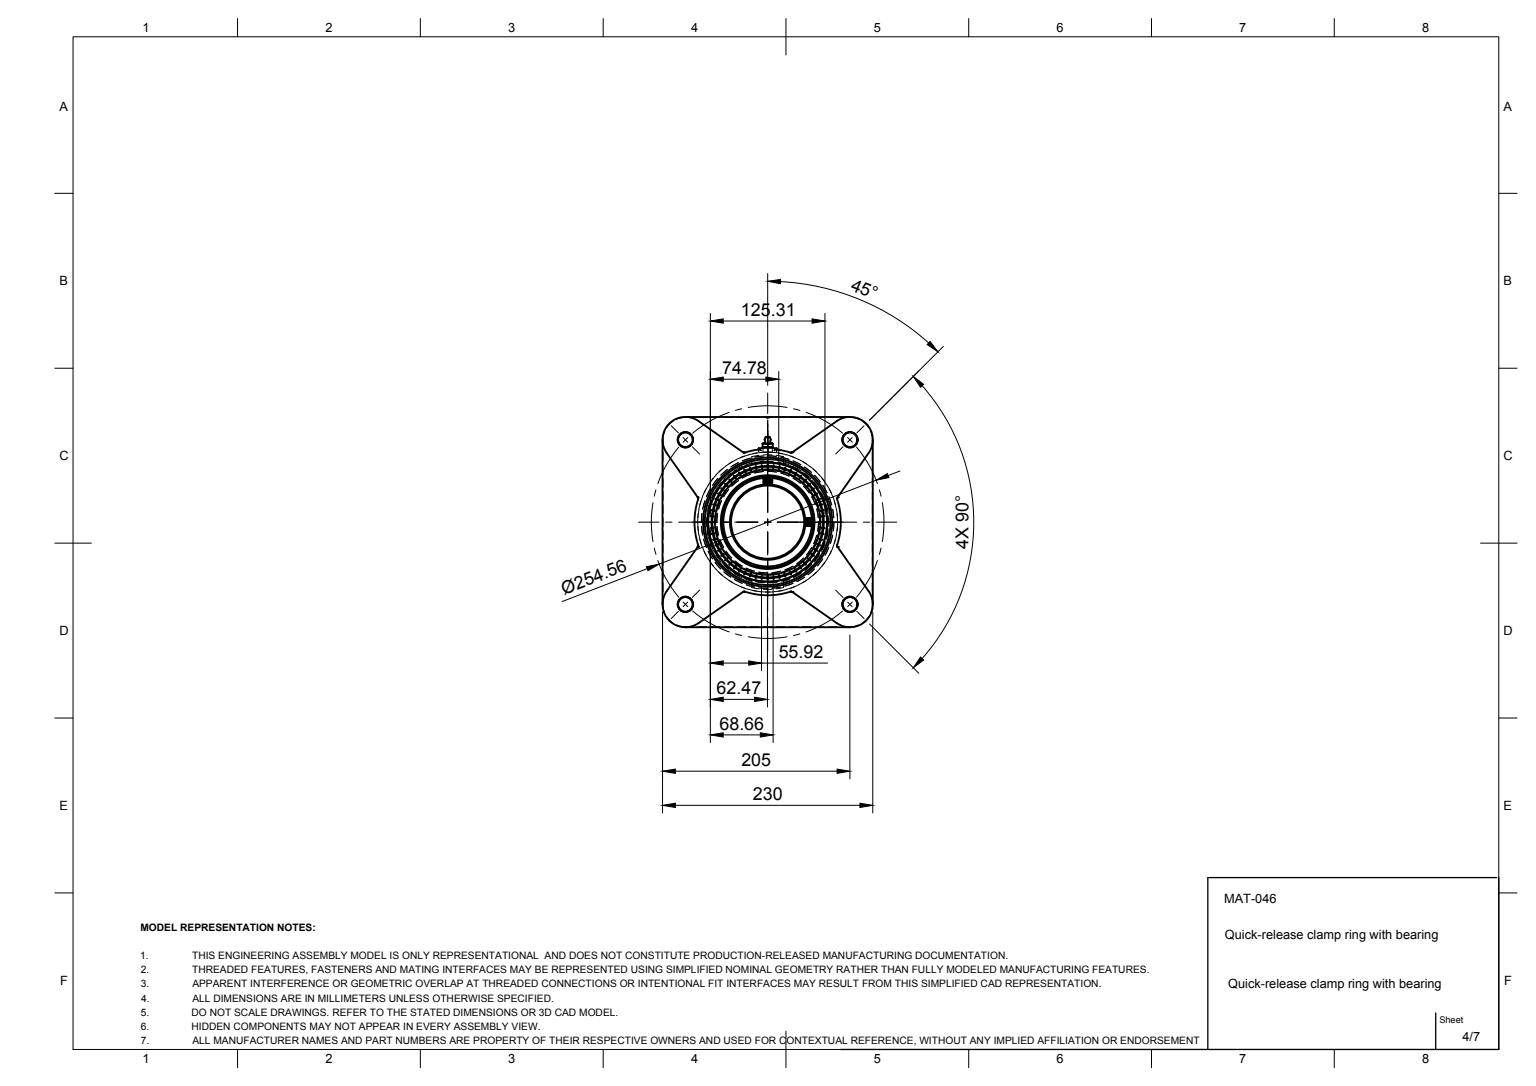
ISO-10303-21;
HEADER;
/* Generated by software containing ST-Developer
 * from STEP Tools, Inc. (www.steptools.com) 
 */

FILE_DESCRIPTION(
/* description */ ('STEP AP214'),
/* implementation_level */ '2;1');

FILE_NAME(
/* name */ 'Quick-release clamp ring with bearing.step',
/* time_stamp */ '2026-11-14T22:16:48-08:00',
/* author */ (''),
/* organization */ (''),
/* preprocessor_version */ 'ST-DEVELOPER v20.2',
/* originating_system */ 'Autodesk Translation Framework v15.17.0.0',
/* authorisation */ '');

FILE_SCHEMA (('AUTOMOTIVE_DESIGN { 1 0 10303 214 3 1 1 }'));
ENDSEC;

DATA;
#10=MECHANICAL_DESIGN_GEOMETRIC_PRESENTATION_REPRESENTATION('',(#5475,#5476,#5477,#5478,#5479,#5480,#5481,#5482,#5483,#5484,#5485,#5486,#5487,#5488,#5489,#5490,#5491,#5492,#5493,#5494,#5495),#276462);
#45=SPHERICAL_SURFACE('',#98960,3.37686862486535);
#46=SPHERICAL_SURFACE('',#110483,1.905);
#47=SPHERICAL_SURFACE('',#110485,1.905);
#48=SPHERICAL_SURFACE('',#110508,0.952499999999998);
#49=SPHERICAL_SURFACE('',#110528,3.17500000000001);
#50=CONICAL_SURFACE('',#98946,5.55625,1.0471975511966);
#51=CONICAL_SURFACE('',#98951,5.55625,1.0471975511966);
#52=CONICAL_SURFACE('',#98954,3.78554799125932,1.22012705768434);
#53=CONICAL_SURFACE('',#98966,2.40973730802039,0.353951387855692);
#54=CONICAL_SURFACE('',#98977,5.55625,1.0471975511966);
#55=CONICAL_SURFACE('',#98978,5.55625,1.0471975511966);
#56=CONICAL_SURFACE('',#98979,5.55625,1.0471975511966);
#57=CONICAL_SURFACE('',#98980,5.55625,1.0471975511966);
#58=CONICAL_SURFACE('',#98981,5.55625,1.0471975511966);
#59=CONICAL_SURFACE('',#98989,5.55625,1.0471975511966);
#60=CONICAL_SURFACE('',#98990,5.55625,1.0471975511966);
#61=CONICAL_SURFACE('',#98991,5.55625,1.0471975511966);
#62=CONICAL_SURFACE('',#98992,5.55625,1.0471975511966);
#63=CONICAL_SURFACE('',#98993,5.55625,1.0471975511966);
#64=CONICAL_SURFACE('',#99119,64.0080199038439,0.558505360638178);
#65=CONICAL_SURFACE('',#99120,62.2224557307631,0.558505360638175);
#66=CONICAL_SURFACE('',#99239,58.6605641730809,0.558505360638184);
#67=CONICAL_SURFACE('',#99359,56.875,0.558505360638184);
#68=CONICAL_SURFACE('',#99369,60.4792282238308,0.523598775598302);
#69=CONICAL_SURFACE('',#99374,61.15975,0.523598775598289);
#70=CONICAL_SURFACE('',#99398,60.4792282238308,0.523598775598302);
#71=CONICAL_SURFACE('',#99403,61.15975,0.523598775598289);
#72=CONICAL_SURFACE('',#99427,60.4792282238308,0.523598775598302);
#73=CONICAL_SURFACE('',#99432,61.15975,0.523598775598289);
#74=CONICAL_SURFACE('',#99456,60.4792282238308,0.523598775598302);
#75=CONICAL_SURFACE('',#99461,61.15975,0.523598775598289);
#76=CONICAL_SURFACE('',#99485,60.4792282238308,0.523598775598302);
#77=CONICAL_SURFACE('',#99490,61.15975,0.523598775598289);
#78=CONICAL_SURFACE('',#99514,60.4792282238308,0.523598775598302);
#79=CONICAL_SURFACE('',#99519,61.15975,0.523598775598289);
#80=CONICAL_SURFACE('',#99543,60.4792282238308,0.523598775598302);
#81=CONICAL_SURFACE('',#99548,61.15975,0.523598775598289);
#82=CONICAL_SURFACE('',#99572,60.4792282238308,0.523598775598302);
#83=CONICAL_SURFACE('',#99577,61.15975,0.523598775598289);
#84=CONICAL_SURFACE('',#99601,60.4792282238308,0.523598775598302);
#85=CONICAL_SURFACE('',#99606,61.15975,0.523598775598289);
#86=CONICAL_SURFACE('',#99630,60.4792282238308,0.523598775598302);
#87=CONICAL_SURFACE('',#99635,61.15975,0.523598775598289);
#88=CONICAL_SURFACE('',#99659,60.4792282238308,0.523598775598302);
#89=CONICAL_SURFACE('',#99664,61.15975,0.523598775598289);
#90=CONICAL_SURFACE('',#99688,60.4792282238308,0.523598775598302);
#91=CONICAL_SURFACE('',#99693,61.15975,0.523598775598289);
#92=CONICAL_SURFACE('',#99717,60.4792282238308,0.523598775598302);
#93=CONICAL_SURFACE('',#99722,61.15975,0.523598775598289);
#94=CONICAL_SURFACE('',#99746,60.4792282238308,0.523598775598302);
#95=CONICAL_SURFACE('',#99751,61.15975,0.523598775598289);
#96=CONICAL_SURFACE('',#99775,60.4792282238308,0.523598775598302);
#97=CONICAL_SURFACE('',#99780,61.15975,0.523598775598289);
#98=CONICAL_SURFACE('',#99804,60.4792282238308,0.523598775598302);
#99=CONICAL_SURFACE('',#99809,61.15975,0.523598775598289);
#100=CONICAL_SURFACE('',#99833,60.4792282238308,0.523598775598302);
#101=CONICAL_SURFACE('',#99838,61.15975,0.523598775598289);
#102=CONICAL_SURFACE('',#99862,60.4792282238308,0.523598775598302);
#103=CONICAL_SURFACE('',#99867,61.15975,0.523598775598289);
#104=CONICAL_SURFACE('',#99891,60.4792282238308,0.523598775598302);
#105=CONICAL_SURFACE('',#99896,61.15975,0.523598775598289);
#106=CONICAL_SURFACE('',#99920,60.4792282238308,0.523598775598302);
#107=CONICAL_SURFACE('',#99925,61.15975,0.523598775598289);
#108=CONICAL_SURFACE('',#99949,60.4792282238308,0.523598775598302);
#109=CONICAL_SURFACE('',#99954,61.15975,0.523598775598289);
#110=CONICAL_SURFACE('',#99978,60.4792282238308,0.523598775598302);
#111=CONICAL_SURFACE('',#99983,61.15975,0.523598775598289);
#112=CONICAL_SURFACE('',#100007,60.4792282238308,0.523598775598302);
#113=CONICAL_SURFACE('',#100012,61.15975,0.523598775598289);
#114=CONICAL_SURFACE('',#100036,60.4792282238308,0.523598775598302);
#115=CONICAL_SURFACE('',#100041,61.15975,0.523598775598289);
#116=CONICAL_SURFACE('',#100065,60.4792282238308,0.523598775598302);
#117=CONICAL_SURFACE('',#100070,61.15975,0.523598775598289);
#118=CONICAL_SURFACE('',#100094,60.4792282238308,0.523598775598302);
#119=CONICAL_SURFACE('',#100099,61.15975,0.523598775598289);
#120=CONICAL_SURFACE('',#100123,60.4792282238308,0.523598775598302);
#121=CONICAL_SURFACE('',#100128,61.15975,0.523598775598289);
#122=CONICAL_SURFACE('',#100152,60.4792282238308,0.523598775598302);
#123=CONICAL_SURFACE('',#100157,61.15975,0.523598775598289);
#124=CONICAL_SURFACE('',#100181,60.4792282238308,0.523598775598302);
#125=CONICAL_SURFACE('',#100186,61.15975,0.523598775598289);
#126=CONICAL_SURFACE('',#100210,60.4792282238308,0.523598775598302);
#127=CONICAL_SURFACE('',#100215,61.15975,0.523598775598289);
#128=CONICAL_SURFACE('',#100239,60.4792282238308,0.523598775598302);
#129=CONICAL_SURFACE('',#100244,61.15975,0.523598775598289);
#130=CONICAL_SURFACE('',#100268,60.4792282238308,0.523598775598302);
#131=CONICAL_SURFACE('',#100273,61.15975,0.523598775598289);
#132=CONICAL_SURFACE('',#100297,60.4792282238308,0.523598775598302);
#133=CONICAL_SURFACE('',#100302,61.15975,0.523598775598289);
#134=CONICAL_SURFACE('',#100326,60.4792282238308,0.523598775598302);
#135=CONICAL_SURFACE('',#100331,61.15975,0.523598775598289);
#136=CONICAL_SURFACE('',#100355,60.4792282238308,0.523598775598302);
#137=CONICAL_SURFACE('',#100360,61.15975,0.523598775598289);
#138=CONICAL_SURFACE('',#100384,60.4792282238308,0.523598775598302);
#139=CONICAL_SURFACE('',#100389,61.15975,0.523598775598289);
#140=CONICAL_SURFACE('',#100413,60.4792282238308,0.523598775598302);
#141=CONICAL_SURFACE('',#100418,61.15975,0.523598775598289);
#142=CONICAL_SURFACE('',#100442,60.4792282238308,0.523598775598302);
#143=CONICAL_SURFACE('',#100447,61.15975,0.523598775598289);
#144=CONICAL_SURFACE('',#100471,60.4792282238308,0.523598775598302);
#145=CONICAL_SURFACE('',#100476,61.15975,0.523598775598289);
#146=CONICAL_SURFACE('',#100500,60.4792282238308,0.523598775598302);
#147=CONICAL_SURFACE('',#100505,61.15975,0.523598775598289);
#148=CONICAL_SURFACE('',#100529,60.4792282238308,0.523598775598302);
#149=CONICAL_SURFACE('',#100534,61.15975,0.523598775598289);
#150=CONICAL_SURFACE('',#100558,60.4792282238308,0.523598775598302);
#151=CONICAL_SURFACE('',#100563,61.15975,0.523598775598289);
#152=CONICAL_SURFACE('',#100587,60.4792282238308,0.523598775598302);
#153=CONICAL_SURFACE('',#100592,61.15975,0.523598775598289);
#154=CONICAL_SURFACE('',#100616,60.4792282238308,0.523598775598302);
#155=CONICAL_SURFACE('',#100621,61.15975,0.523598775598289);
#156=CONICAL_SURFACE('',#100645,60.4792282238308,0.523598775598302);
#157=CONICAL_SURFACE('',#100650,61.15975,0.523598775598289);
#158=CONICAL_SURFACE('',#100674,60.4792282238308,0.523598775598302);
#159=CONICAL_SURFACE('',#100679,61.15975,0.523598775598289);
#160=CONICAL_SURFACE('',#100703,60.4792282238308,0.523598775598302);
#161=CONICAL_SURFACE('',#100708,61.15975,0.523598775598289);
#162=CONICAL_SURFACE('',#100732,60.4792282238308,0.523598775598302);
#163=CONICAL_SURFACE('',#100737,61.15975,0.523598775598289);
#164=CONICAL_SURFACE('',#100761,60.4792282238308,0.523598775598302);
#165=CONICAL_SURFACE('',#100766,61.15975,0.523598775598289);
#166=CONICAL_SURFACE('',#100790,60.4792282238308,0.523598775598302);
#167=CONICAL_SURFACE('',#100795,61.15975,0.523598775598289);
#168=CONICAL_SURFACE('',#100819,60.4792282238308,0.523598775598302);
#169=CONICAL_SURFACE('',#100824,61.15975,0.523598775598289);
#170=CONICAL_SURFACE('',#100848,60.4792282238308,0.523598775598302);
#171=CONICAL_SURFACE('',#100853,61.15975,0.523598775598289);
#172=CONICAL_SURFACE('',#100877,60.4792282238308,0.523598775598302);
#173=CONICAL_SURFACE('',#100882,61.15975,0.523598775598289);
#174=CONICAL_SURFACE('',#100906,60.4792282238308,0.523598775598302);
#175=CONICAL_SURFACE('',#100911,61.15975,0.523598775598289);
#176=CONICAL_SURFACE('',#100935,60.4792282238308,0.523598775598302);
#177=CONICAL_SURFACE('',#100940,61.15975,0.523598775598289);
#178=CONICAL_SURFACE('',#100964,60.4792282238308,0.523598775598302);
#179=CONICAL_SURFACE('',#100969,61.15975,0.523598775598289);
#180=CONICAL_SURFACE('',#100993,60.4792282238308,0.523598775598302);
#181=CONICAL_SURFACE('',#100998,61.15975,0.523598775598289);
#182=CONICAL_SURFACE('',#101022,60.4792282238308,0.523598775598302);
#183=CONICAL_SURFACE('',#101027,61.15975,0.523598775598289);
#184=CONICAL_SURFACE('',#101051,60.4792282238308,0.523598775598302);
#185=CONICAL_SURFACE('',#101056,61.15975,0.523598775598289);
#186=CONICAL_SURFACE('',#101081,60.4792282238308,0.523598775598302);
#187=CONICAL_SURFACE('',#101086,61.15975,0.523598775598289);
#188=CONICAL_SURFACE('',#104673,64.0080199038439,0.558505360638178);
#189=CONICAL_SURFACE('',#104674,62.2224557307631,0.558505360638175);
#190=CONICAL_SURFACE('',#104793,58.6605641730809,0.558505360638184);
#191=CONICAL_SURFACE('',#104913,56.875,0.558505360638184);
#192=CONICAL_SURFACE('',#104923,60.4792282238308,0.523598775598302);
#193=CONICAL_SURFACE('',#104928,61.15975,0.523598775598289);
#194=CONICAL_SURFACE('',#104952,60.4792282238308,0.523598775598302);
#195=CONICAL_SURFACE('',#104957,61.15975,0.523598775598289);
#196=CONICAL_SURFACE('',#104981,60.4792282238308,0.523598775598302);
#197=CONICAL_SURFACE('',#104986,61.15975,0.523598775598289);
#198=CONICAL_SURFACE('',#105010,60.4792282238308,0.523598775598302);
#199=CONICAL_SURFACE('',#105015,61.15975,0.523598775598289);
#200=CONICAL_SURFACE('',#105039,60.4792282238308,0.523598775598302);
#201=CONICAL_SURFACE('',#105044,61.15975,0.523598775598289);
#202=CONICAL_SURFACE('',#105068,60.4792282238308,0.523598775598302);
#203=CONICAL_SURFACE('',#105073,61.15975,0.523598775598289);
#204=CONICAL_SURFACE('',#105097,60.4792282238308,0.523598775598302);
#205=CONICAL_SURFACE('',#105102,61.15975,0.523598775598289);
#206=CONICAL_SURFACE('',#105126,60.4792282238308,0.523598775598302);
#207=CONICAL_SURFACE('',#105131,61.15975,0.523598775598289);
#208=CONICAL_SURFACE('',#105155,60.4792282238308,0.523598775598302);
#209=CONICAL_SURFACE('',#105160,61.15975,0.523598775598289);
#210=CONICAL_SURFACE('',#105184,60.4792282238308,0.523598775598302);
#211=CONICAL_SURFACE('',#105189,61.15975,0.523598775598289);
#212=CONICAL_SURFACE('',#105213,60.4792282238308,0.523598775598302);
#213=CONICAL_SURFACE('',#105218,61.15975,0.523598775598289);
#214=CONICAL_SURFACE('',#105242,60.4792282238308,0.523598775598302);
#215=CONICAL_SURFACE('',#105247,61.15975,0.523598775598289);
#216=CONICAL_SURFACE('',#105271,60.4792282238308,0.523598775598302);
#217=CONICAL_SURFACE('',#105276,61.15975,0.523598775598289);
#218=CONICAL_SURFACE('',#105300,60.4792282238308,0.523598775598302);
#219=CONICAL_SURFACE('',#105305,61.15975,0.523598775598289);
#220=CONICAL_SURFACE('',#105329,60.4792282238308,0.523598775598302);
#221=CONICAL_SURFACE('',#105334,61.15975,0.523598775598289);
#222=CONICAL_SURFACE('',#105358,60.4792282238308,0.523598775598302);
#223=CONICAL_SURFACE('',#105363,61.15975,0.523598775598289);
#224=CONICAL_SURFACE('',#105387,60.4792282238308,0.523598775598302);
#225=CONICAL_SURFACE('',#105392,61.15975,0.523598775598289);
#226=CONICAL_SURFACE('',#105416,60.4792282238308,0.523598775598302);
#227=CONICAL_SURFACE('',#105421,61.15975,0.523598775598289);
#228=CONICAL_SURFACE('',#105445,60.4792282238308,0.523598775598302);
#229=CONICAL_SURFACE('',#105450,61.15975,0.523598775598289);
#230=CONICAL_SURFACE('',#105474,60.4792282238308,0.523598775598302);
#231=CONICAL_SURFACE('',#105479,61.15975,0.523598775598289);
#232=CONICAL_SURFACE('',#105503,60.4792282238308,0.523598775598302);
#233=CONICAL_SURFACE('',#105508,61.15975,0.523598775598289);
#234=CONICAL_SURFACE('',#105532,60.4792282238308,0.523598775598302);
#235=CONICAL_SURFACE('',#105537,61.15975,0.523598775598289);
#236=CONICAL_SURFACE('',#105561,60.4792282238308,0.523598775598302);
#237=CONICAL_SURFACE('',#105566,61.15975,0.523598775598289);
#238=CONICAL_SURFACE('',#105590,60.4792282238308,0.523598775598302);
#239=CONICAL_SURFACE('',#105595,61.15975,0.523598775598289);
#240=CONICAL_SURFACE('',#105619,60.4792282238308,0.523598775598302);
#241=CONICAL_SURFACE('',#105624,61.15975,0.523598775598289);
#242=CONICAL_SURFACE('',#105648,60.4792282238308,0.523598775598302);
#243=CONICAL_SURFACE('',#105653,61.15975,0.523598775598289);
#244=CONICAL_SURFACE('',#105677,60.4792282238308,0.523598775598302);
#245=CONICAL_SURFACE('',#105682,61.15975,0.523598775598289);
#246=CONICAL_SURFACE('',#105706,60.4792282238308,0.523598775598302);
#247=CONICAL_SURFACE('',#105711,61.15975,0.523598775598289);
#248=CONICAL_SURFACE('',#105735,60.4792282238308,0.523598775598302);
#249=CONICAL_SURFACE('',#105740,61.15975,0.523598775598289);
#250=CONICAL_SURFACE('',#105764,60.4792282238308,0.523598775598302);
#251=CONICAL_SURFACE('',#105769,61.15975,0.523598775598289);
#252=CONICAL_SURFACE('',#105793,60.4792282238308,0.523598775598302);
#253=CONICAL_SURFACE('',#105798,61.15975,0.523598775598289);
#254=CONICAL_SURFACE('',#105822,60.4792282238308,0.523598775598302);
#255=CONICAL_SURFACE('',#105827,61.15975,0.523598775598289);
#256=CONICAL_SURFACE('',#105851,60.4792282238308,0.523598775598302);
#257=CONICAL_SURFACE('',#105856,61.15975,0.523598775598289);
#258=CONICAL_SURFACE('',#105880,60.4792282238308,0.523598775598302);
#259=CONICAL_SURFACE('',#105885,61.15975,0.523598775598289);
#260=CONICAL_SURFACE('',#105909,60.4792282238308,0.523598775598302);
#261=CONICAL_SURFACE('',#105914,61.15975,0.523598775598289);
#262=CONICAL_SURFACE('',#105938,60.4792282238308,0.523598775598302);
#263=CONICAL_SURFACE('',#105943,61.15975,0.523598775598289);
#264=CONICAL_SURFACE('',#105967,60.4792282238308,0.523598775598302);
#265=CONICAL_SURFACE('',#105972,61.15975,0.523598775598289);
#266=CONICAL_SURFACE('',#105996,60.4792282238308,0.523598775598302);
#267=CONICAL_SURFACE('',#106001,61.15975,0.523598775598289);
#268=CONICAL_SURFACE('',#106025,60.4792282238308,0.523598775598302);
#269=CONICAL_SURFACE('',#106030,61.15975,0.523598775598289);
#270=CONICAL_SURFACE('',#106054,60.4792282238308,0.523598775598302);
#271=CONICAL_SURFACE('',#106059,61.15975,0.523598775598289);
#272=CONICAL_SURFACE('',#106083,60.4792282238308,0.523598775598302);
#273=CONICAL_SURFACE('',#106088,61.15975,0.523598775598289);
#274=CONICAL_SURFACE('',#106112,60.4792282238308,0.523598775598302);
#275=CONICAL_SURFACE('',#106117,61.15975,0.523598775598289);
#276=CONICAL_SURFACE('',#106141,60.4792282238308,0.523598775598302);
#277=CONICAL_SURFACE('',#106146,61.15975,0.523598775598289);
#278=CONICAL_SURFACE('',#106170,60.4792282238308,0.523598775598302);
#279=CONICAL_SURFACE('',#106175,61.15975,0.523598775598289);
#280=CONICAL_SURFACE('',#106199,60.4792282238308,0.523598775598302);
#281=CONICAL_SURFACE('',#106204,61.15975,0.523598775598289);
#282=CONICAL_SURFACE('',#106228,60.4792282238308,0.523598775598302);
#283=CONICAL_SURFACE('',#106233,61.15975,0.523598775598289);
#284=CONICAL_SURFACE('',#106257,60.4792282238308,0.523598775598302);
#285=CONICAL_SURFACE('',#106262,61.15975,0.523598775598289);
#286=CONICAL_SURFACE('',#106286,60.4792282238308,0.523598775598302);
#287=CONICAL_SURFACE('',#106291,61.15975,0.523598775598289);
#288=CONICAL_SURFACE('',#106315,60.4792282238308,0.523598775598302);
#289=CONICAL_SURFACE('',#106320,61.15975,0.523598775598289);
#290=CONICAL_SURFACE('',#106344,60.4792282238308,0.523598775598302);
#291=CONICAL_SURFACE('',#106349,61.15975,0.523598775598289);
#292=CONICAL_SURFACE('',#106373,60.4792282238308,0.523598775598302);
#293=CONICAL_SURFACE('',#106378,61.15975,0.523598775598289);
#294=CONICAL_SURFACE('',#106402,60.4792282238308,0.523598775598302);
#295=CONICAL_SURFACE('',#106407,61.15975,0.523598775598289);
#296=CONICAL_SURFACE('',#106431,60.4792282238308,0.523598775598302);
#297=CONICAL_SURFACE('',#106436,61.15975,0.523598775598289);
#298=CONICAL_SURFACE('',#106460,60.4792282238308,0.523598775598302);
#299=CONICAL_SURFACE('',#106465,61.15975,0.523598775598289);
#300=CONICAL_SURFACE('',#106489,60.4792282238308,0.523598775598302);
#301=CONICAL_SURFACE('',#106494,61.15975,0.523598775598289);
#302=CONICAL_SURFACE('',#106518,60.4792282238308,0.523598775598302);
#303=CONICAL_SURFACE('',#106523,61.15975,0.523598775598289);
#304=CONICAL_SURFACE('',#106547,60.4792282238308,0.523598775598302);
#305=CONICAL_SURFACE('',#106552,61.15975,0.523598775598289);
#306=CONICAL_SURFACE('',#106576,60.4792282238308,0.523598775598302);
#307=CONICAL_SURFACE('',#106581,61.15975,0.523598775598289);
#308=CONICAL_SURFACE('',#106605,60.4792282238308,0.523598775598302);
#309=CONICAL_SURFACE('',#106610,61.15975,0.523598775598289);
#310=CONICAL_SURFACE('',#106635,60.4792282238308,0.523598775598302);
#311=CONICAL_SURFACE('',#106640,61.15975,0.523598775598289);
#312=CONICAL_SURFACE('',#110283,80.,0.122173047639603);
#313=CONICAL_SURFACE('',#110573,56.2993860673093,0.55850536063818);
#314=CONICAL_SURFACE('',#110574,57.8669800961561,0.558505360638184);
#315=CONICAL_SURFACE('',#110605,4.74980000000001,0.78539816339745);
#316=CONICAL_SURFACE('',#110610,3.98780000000001,0.785398163397452);
#317=CONICAL_SURFACE('',#110625,2.7496306570156,0.78539816339745);
#318=CONICAL_SURFACE('',#110626,2.7496306570156,0.78539816339745);
#319=CONICAL_SURFACE('',#110627,2.7496306570156,0.78539816339745);
#320=CONICAL_SURFACE('',#110628,2.7496306570156,0.78539816339745);
#321=CONICAL_SURFACE('',#110629,2.7496306570156,0.78539816339745);
#322=CONICAL_SURFACE('',#110630,2.7496306570156,0.78539816339745);
#323=CONICAL_SURFACE('',#110657,4.74980000000001,0.78539816339745);
#324=CONICAL_SURFACE('',#110662,3.98780000000001,0.785398163397452);
#325=CONICAL_SURFACE('',#110677,2.7496306570156,0.78539816339745);
#326=CONICAL_SURFACE('',#110678,2.7496306570156,0.78539816339745);
#327=CONICAL_SURFACE('',#110679,2.7496306570156,0.78539816339745);
#328=CONICAL_SURFACE('',#110680,2.7496306570156,0.78539816339745);
#329=CONICAL_SURFACE('',#110681,2.7496306570156,0.78539816339745);
#330=CONICAL_SURFACE('',#110682,2.7496306570156,0.78539816339745);
#331=CONICAL_SURFACE('',#110691,40.,0.698131700797724);
#332=CONICAL_SURFACE('',#110694,40.,0.698131700797741);
#333=CONICAL_SURFACE('',#110698,48.4864729374055,0.872664625997157);
#334=CONICAL_SURFACE('',#110701,48.4864729374054,0.872664625997163);
#338=ELLIPSE('',#99385,0.599370291563849,0.555629413547353);
#339=ELLIPSE('',#99386,0.599370913936212,0.555630771247294);
#340=ELLIPSE('',#99388,0.239805704052526,0.222043163089743);
#341=ELLIPSE('',#99389,0.239805889069737,0.222043643391604);
#342=ELLIPSE('',#99391,0.239805882895812,0.222043378689669);
#343=ELLIPSE('',#99392,0.239805697268466,0.22204289662789);
#344=ELLIPSE('',#99414,0.599370913936647,0.555630771248094);
#345=ELLIPSE('',#99415,0.599370291565284,0.555629413550211);
#346=ELLIPSE('',#99417,0.239805889071228,0.222043643394759);
#347=ELLIPSE('',#99418,0.239805704054646,0.222043163093994);
#348=ELLIPSE('',#99420,0.239805697269572,0.222042896630273);
#349=ELLIPSE('',#99421,0.239805882893992,0.222043378685954);
#350=ELLIPSE('',#99443,0.599370913939605,0.555630771254153);
#351=ELLIPSE('',#99444,0.599370291563661,0.555629413546882);
#352=ELLIPSE('',#99446,0.23980588906817,0.222043643388294);
#353=ELLIPSE('',#99447,0.239805704052944,0.222043163090554);
#354=ELLIPSE('',#99449,0.239805697268366,0.222042896627733);
#355=ELLIPSE('',#99450,0.239805882894834,0.222043378687724);
#356=ELLIPSE('',#99472,0.599370913938154,0.55563077125104);
#357=ELLIPSE('',#99473,0.59937029156276,0.555629413545193);
#358=ELLIPSE('',#99475,0.239805889066608,0.222043643385116);
#359=ELLIPSE('',#99476,0.239805704053829,0.22204316309239);
#360=ELLIPSE('',#99478,0.239805697267153,0.222042896625171);
#361=ELLIPSE('',#99479,0.239805882894158,0.222043378686371);
#362=ELLIPSE('',#99501,0.599370913936745,0.55563077124828);
#363=ELLIPSE('',#99502,0.599370291565539,0.555629413550565);
#364=ELLIPSE('',#99504,0.239805889071284,0.222043643394696);
#365=ELLIPSE('',#99505,0.239805704051857,0.222043163088228);
#366=ELLIPSE('',#99507,0.239805697269279,0.222042896629737);
#367=ELLIPSE('',#99508,0.239805882895886,0.222043378689775);
#368=ELLIPSE('',#99530,0.599370913935051,0.555630771244647);
#369=ELLIPSE('',#99531,0.599370291563104,0.555629413545832);
#370=ELLIPSE('',#99533,0.239805889067115,0.222043643386276);
#371=ELLIPSE('',#99534,0.239805704053193,0.222043163090947);
#372=ELLIPSE('',#99536,0.239805697268009,0.222042896626989);
#373=ELLIPSE('',#99537,0.239805882895764,0.222043378689474);
#374=ELLIPSE('',#99559,0.599370913937216,0.555630771249188);
#375=ELLIPSE('',#99560,0.599370291563396,0.555629413546297);
#376=ELLIPSE('',#99562,0.239805889067743,0.222043643387537);
#377=ELLIPSE('',#99563,0.239805704055465,0.222043163095698);
#378=ELLIPSE('',#99565,0.239805697269418,0.222042896629816);
#379=ELLIPSE('',#99566,0.239805882894163,0.222043378686227);
#380=ELLIPSE('',#99588,0.599370913937631,0.555630771249981);
#381=ELLIPSE('',#99589,0.599370291563643,0.555629413546836);
#382=ELLIPSE('',#99591,0.239805889070487,0.222043643393142);
#383=ELLIPSE('',#99592,0.239805704052451,0.222043163089509);
#384=ELLIPSE('',#99594,0.239805697268519,0.222042896628072);
#385=ELLIPSE('',#99595,0.239805882895209,0.222043378688398);
#386=ELLIPSE('',#99617,0.599370913936379,0.555630771247499);
#387=ELLIPSE('',#99618,0.599370291564538,0.55562941354869);
#388=ELLIPSE('',#99620,0.239805889068884,0.222043643389916);
#389=ELLIPSE('',#99621,0.239805704050981,0.222043163086484);
#390=ELLIPSE('',#99623,0.239805697268942,0.222042896628818);
#391=ELLIPSE('',#99624,0.239805882895923,0.222043378689984);
#392=ELLIPSE('',#99646,0.59937091393689,0.555630771248566);
#393=ELLIPSE('',#99647,0.599370291565025,0.555629413549741);
#394=ELLIPSE('',#99649,0.239805889069351,0.222043643390883);
#395=ELLIPSE('',#99650,0.239805704051609,0.222043163087727);
#396=ELLIPSE('',#99652,0.239805697270396,0.222042896631823);
#397=ELLIPSE('',#99653,0.239805882896325,0.222043378690807);
#398=ELLIPSE('',#99675,0.599370913934826,0.555630771244343);
#399=ELLIPSE('',#99676,0.599370291564194,0.555629413547986);
#400=ELLIPSE('',#99678,0.239805889068253,0.222043643388627);
#401=ELLIPSE('',#99679,0.239805704053178,0.222043163090936);
#402=ELLIPSE('',#99681,0.239805697270034,0.22204289663126);
#403=ELLIPSE('',#99682,0.239805882893466,0.222043378684868);
#404=ELLIPSE('',#99704,0.59937091393641,0.55563077124766);
#405=ELLIPSE('',#99705,0.599370291564805,0.555629413549147);
#406=ELLIPSE('',#99707,0.239805889072066,0.222043643396362);
#407=ELLIPSE('',#99708,0.239805704052236,0.22204316308897);
#408=ELLIPSE('',#99710,0.23980569726934,0.222042896629804);
#409=ELLIPSE('',#99711,0.239805882895727,0.222043378689497);
#410=ELLIPSE('',#99733,0.599370913936658,0.555630771248057);
#411=ELLIPSE('',#99734,0.599370291562746,0.555629413545113);
#412=ELLIPSE('',#99736,0.239805889070185,0.222043643392531);
#413=ELLIPSE('',#99737,0.239805704053294,0.222043163091287);
#414=ELLIPSE('',#99739,0.239805697268977,0.222042896628983);
#415=ELLIPSE('',#99740,0.239805882896423,0.222043378690919);
#416=ELLIPSE('',#99762,0.59937091393644,0.555630771247594);
#417=ELLIPSE('',#99763,0.599370291561981,0.55562941354343);
#418=ELLIPSE('',#99765,0.239805889071035,0.222043643394202);
#419=ELLIPSE('',#99766,0.239805704052008,0.222043163088609);
#420=ELLIPSE('',#99768,0.239805697269648,0.222042896630424);
#421=ELLIPSE('',#99769,0.239805882895413,0.222043378688915);
#422=ELLIPSE('',#99791,0.599370913936381,0.555630771247481);
#423=ELLIPSE('',#99792,0.599370291564673,0.555629413548984);
#424=ELLIPSE('',#99794,0.239805889068991,0.222043643390099);
#425=ELLIPSE('',#99795,0.239805704053787,0.222043163092241);
#426=ELLIPSE('',#99797,0.239805697268383,0.222042896627734);
#427=ELLIPSE('',#99798,0.239805882893284,0.222043378684528);
#428=ELLIPSE('',#99820,0.599370913934144,0.555630771243034);
#429=ELLIPSE('',#99821,0.599370291566355,0.55562941355229);
#430=ELLIPSE('',#99823,0.239805889070614,0.222043643393421);
#431=ELLIPSE('',#99824,0.239805704053183,0.22204316309096);
#432=ELLIPSE('',#99826,0.239805697269667,0.222042896630443);
#433=ELLIPSE('',#99827,0.239805882894449,0.222043378686902);
#434=ELLIPSE('',#99849,0.599370913938034,0.555630771250937);
#435=ELLIPSE('',#99850,0.599370291564758,0.555629413549118);
#436=ELLIPSE('',#99852,0.239805889071379,0.222043643395086);
#437=ELLIPSE('',#99853,0.239805704051962,0.222043163088545);
#438=ELLIPSE('',#99855,0.239805697269236,0.222042896629485);
#439=ELLIPSE('',#99856,0.239805882895064,0.222043378688177);
#440=ELLIPSE('',#99878,0.599370913936816,0.555630771248509);
#441=ELLIPSE('',#99879,0.599370291562686,0.555629413544951);
#442=ELLIPSE('',#99881,0.239805889072334,0.222043643396888);
#443=ELLIPSE('',#99882,0.239805704051859,0.222043163088407);
#444=ELLIPSE('',#99884,0.239805697267012,0.222042896625054);
#445=ELLIPSE('',#99885,0.239805882894425,0.2220433786868);
#446=ELLIPSE('',#99907,0.599370913937916,0.555630771250686);
#447=ELLIPSE('',#99908,0.599370291561844,0.555629413543086);
#448=ELLIPSE('',#99910,0.239805889071215,0.222043643394601);
#449=ELLIPSE('',#99911,0.239805704052586,0.222043163089754);
#450=ELLIPSE('',#99913,0.239805697269129,0.222042896629312);
#451=ELLIPSE('',#99914,0.239805882895691,0.222043378689463);
#452=ELLIPSE('',#99936,0.599370913935739,0.555630771246241);
#453=ELLIPSE('',#99937,0.599370291565713,0.555629413551048);
#454=ELLIPSE('',#99939,0.239805889070012,0.222043643392159);
#455=ELLIPSE('',#99940,0.239805704055269,0.222043163095158);
#456=ELLIPSE('',#99942,0.239805697269079,0.22204289662915);
#457=ELLIPSE('',#99943,0.239805882893285,0.222043378684511);
#458=ELLIPSE('',#99965,0.5993709139378,0.555630771250281);
#459=ELLIPSE('',#99966,0.599370291564487,0.555629413548595);
#460=ELLIPSE('',#99968,0.239805889067021,0.222043643386073);
#461=ELLIPSE('',#99969,0.23980570405032,0.222043163085142);
#462=ELLIPSE('',#99971,0.239805697268822,0.222042896628661);
#463=ELLIPSE('',#99972,0.239805882895231,0.222043378688526);
#464=ELLIPSE('',#99994,0.599370913939247,0.555630771253286);
#465=ELLIPSE('',#99995,0.599370291564407,0.555629413548329);
#466=ELLIPSE('',#99997,0.239805889070316,0.22204364339277);
#467=ELLIPSE('',#99998,0.239805704051555,0.222043163087709);
#468=ELLIPSE('',#100000,0.23980569726812,0.222042896627117);
#469=ELLIPSE('',#100001,0.239805882894233,0.222043378686419);
#470=ELLIPSE('',#100023,0.599370913938812,0.555630771252417);
#471=ELLIPSE('',#100024,0.599370291562947,0.555629413545446);
#472=ELLIPSE('',#100026,0.239805889071155,0.222043643394403);
#473=ELLIPSE('',#100027,0.239805704051147,0.222043163086946);
#474=ELLIPSE('',#100029,0.239805697268128,0.222042896627196);
#475=ELLIPSE('',#100030,0.239805882895692,0.222043378689339);
#476=ELLIPSE('',#100052,0.599370913937403,0.555630771249492);
#477=ELLIPSE('',#100053,0.599370291564698,0.555629413548919);
#478=ELLIPSE('',#100055,0.239805889070393,0.222043643392999);
#479=ELLIPSE('',#100056,0.23980570405366,0.222043163091951);
#480=ELLIPSE('',#100058,0.239805697268035,0.222042896626935);
#481=ELLIPSE('',#100059,0.239805882893378,0.222043378684874);
#482=ELLIPSE('',#100081,0.599370913937259,0.555630771249076);
#483=ELLIPSE('',#100082,0.599370291562252,0.555629413544049);
#484=ELLIPSE('',#100084,0.239805889069568,0.22204364339119);
#485=ELLIPSE('',#100085,0.239805704052158,0.222043163089004);
#486=ELLIPSE('',#100087,0.239805697269194,0.222042896629392);
#487=ELLIPSE('',#100088,0.239805882896074,0.222043378690194);
#488=ELLIPSE('',#100110,0.599370913936119,0.555630771246838);
#489=ELLIPSE('',#100111,0.599370291565987,0.555629413551609);
#490=ELLIPSE('',#100113,0.239805889068597,0.222043643389295);
#491=ELLIPSE('',#100114,0.239805704052637,0.222043163089979);
#492=ELLIPSE('',#100116,0.239805697268707,0.222042896628356);
#493=ELLIPSE('',#100117,0.239805882896297,0.222043378690738);
#494=ELLIPSE('',#100139,0.59937091393601,0.555630771246725);
#495=ELLIPSE('',#100140,0.599370291562778,0.55562941354504);
#496=ELLIPSE('',#100142,0.239805889066727,0.222043643385389);
#497=ELLIPSE('',#100143,0.239805704051771,0.222043163088038);
#498=ELLIPSE('',#100145,0.239805697269733,0.222042896630494);
#499=ELLIPSE('',#100146,0.239805882893609,0.222043378685193);
#500=ELLIPSE('',#100168,0.599370913937713,0.555630771250117);
#501=ELLIPSE('',#100169,0.599370291561973,0.555629413543533);
#502=ELLIPSE('',#100171,0.239805889070764,0.222043643393701);
#503=ELLIPSE('',#100172,0.23980570405167,0.222043163087902);
#504=ELLIPSE('',#100174,0.239805697268835,0.222042896628737);
#505=ELLIPSE('',#100175,0.239805882892975,0.222043378683968);
#506=ELLIPSE('',#100197,0.599370913937063,0.555630771248936);
#507=ELLIPSE('',#100198,0.599370291565828,0.555629413551464);
#508=ELLIPSE('',#100200,0.239805889070764,0.222043643393715);
#509=ELLIPSE('',#100201,0.239805704049691,0.222043163083863);
#510=ELLIPSE('',#100203,0.239805697267964,0.222042896626842);
#511=ELLIPSE('',#100204,0.239805882894855,0.222043378687784);
#512=ELLIPSE('',#100226,0.599370913936629,0.555630771247946);
#513=ELLIPSE('',#100227,0.599370291564561,0.555629413548711);
#514=ELLIPSE('',#100229,0.239805889071998,0.222043643396255);
#515=ELLIPSE('',#100230,0.239805704055809,0.222043163096413);
#516=ELLIPSE('',#100232,0.239805697268767,0.222042896628554);
#517=ELLIPSE('',#100233,0.239805882895225,0.222043378688595);
#518=ELLIPSE('',#100255,0.599370913935967,0.555630771246675);
#519=ELLIPSE('',#100256,0.599370291564349,0.555629413548285);
#520=ELLIPSE('',#100258,0.239805889071902,0.222043643396007);
#521=ELLIPSE('',#100259,0.239805704053452,0.222043163091509);
#522=ELLIPSE('',#100261,0.239805697270489,0.222042896632057);
#523=ELLIPSE('',#100262,0.239805882894835,0.222043378687749);
#524=ELLIPSE('',#100284,0.599370913939248,0.555630771253297);
#525=ELLIPSE('',#100285,0.599370291563863,0.555629413547267);
#526=ELLIPSE('',#100287,0.239805889070602,0.222043643393333);
#527=ELLIPSE('',#100288,0.239805704052742,0.222043163090224);
#528=ELLIPSE('',#100290,0.239805697268792,0.222042896628584);
#529=ELLIPSE('',#100291,0.239805882894068,0.222043378686095);
#530=ELLIPSE('',#100313,0.599370913936219,0.555630771247178);
#531=ELLIPSE('',#100314,0.59937029156409,0.555629413547847);
#532=ELLIPSE('',#100316,0.239805889069997,0.222043643392213);
#533=ELLIPSE('',#100317,0.239805704052893,0.222043163090333);
#534=ELLIPSE('',#100319,0.239805697270079,0.222042896631273);
#535=ELLIPSE('',#100320,0.239805882895664,0.22204337868938);
#536=ELLIPSE('',#100342,0.599370913936394,0.555630771247526);
#537=ELLIPSE('',#100343,0.599370291564918,0.55562941354947);
#538=ELLIPSE('',#100345,0.239805889068249,0.222043643388543);
#539=ELLIPSE('',#100346,0.239805704052389,0.222043163089305);
#540=ELLIPSE('',#100348,0.239805697268477,0.222042896628032);
#541=ELLIPSE('',#100349,0.239805882896082,0.22204337869017);
#542=ELLIPSE('',#100371,0.599370913936562,0.555630771247845);
#543=ELLIPSE('',#100372,0.599370291564012,0.555629413547624);
#544=ELLIPSE('',#100374,0.23980588906986,0.222043643391904);
#545=ELLIPSE('',#100375,0.239805704051993,0.222043163088566);
#546=ELLIPSE('',#100377,0.239805697267169,0.222042896625307);
#547=ELLIPSE('',#100378,0.239805882896219,0.222043378690621);
#548=ELLIPSE('',#100400,0.599370913937084,0.555630771249008);
#549=ELLIPSE('',#100401,0.599370291564365,0.55562941354837);
#550=ELLIPSE('',#100403,0.239805889067811,0.222043643387605);
#551=ELLIPSE('',#100404,0.239805704053666,0.222043163091892);
#552=ELLIPSE('',#100406,0.239805697268621,0.222042896628293);
#553=ELLIPSE('',#100407,0.239805882895389,0.222043378688838);
#554=ELLIPSE('',#100429,0.599370913937905,0.555630771250672);
#555=ELLIPSE('',#100430,0.599370291564906,0.555629413549538);
#556=ELLIPSE('',#100432,0.23980588906824,0.222043643388556);
#557=ELLIPSE('',#100433,0.239805704052944,0.222043163090377);
#558=ELLIPSE('',#100435,0.239805697269778,0.222042896630677);
#559=ELLIPSE('',#100436,0.239805882894411,0.222043378686794);
#560=ELLIPSE('',#100458,0.599370913936309,0.555630771247401);
#561=ELLIPSE('',#100459,0.59937029156245,0.555629413544366);
#562=ELLIPSE('',#100461,0.239805889070967,0.222043643394125);
#563=ELLIPSE('',#100462,0.239805704052184,0.222043163088965);
#564=ELLIPSE('',#100464,0.239805697269359,0.222042896629841);
#565=ELLIPSE('',#100465,0.239805882895676,0.222043378689375);
#566=ELLIPSE('',#100487,0.599370913938664,0.555630771252272);
#567=ELLIPSE('',#100488,0.599370291563739,0.555629413547119);
#568=ELLIPSE('',#100490,0.239805889069012,0.222043643390162);
#569=ELLIPSE('',#100491,0.239805704051928,0.222043163088434);
#570=ELLIPSE('',#100493,0.239805697270961,0.222042896633077);
#571=ELLIPSE('',#100494,0.239805882894207,0.222043378686478);
#572=ELLIPSE('',#100516,0.599370913935456,0.555630771245561);
#573=ELLIPSE('',#100517,0.599370291564729,0.555629413549092);
#574=ELLIPSE('',#100519,0.239805889068523,0.222043643389264);
#575=ELLIPSE('',#100520,0.239805704050355,0.222043163085222);
#576=ELLIPSE('',#100522,0.239805697270177,0.222042896631395);
#577=ELLIPSE('',#100523,0.239805882895827,0.222043378689797);
#578=ELLIPSE('',#100545,0.599370913936989,0.55563077124874);
#579=ELLIPSE('',#100546,0.599370291565551,0.555629413550739);
#580=ELLIPSE('',#100548,0.239805889072759,0.222043643397765);
#581=ELLIPSE('',#100549,0.239805704052168,0.222043163088979);
#582=ELLIPSE('',#100551,0.239805697270002,0.222042896630934);
#583=ELLIPSE('',#100552,0.239805882896146,0.222043378690432);
#584=ELLIPSE('',#100574,0.599370913936148,0.555630771247047);
#585=ELLIPSE('',#100575,0.599370291563679,0.555629413546916);
#586=ELLIPSE('',#100577,0.239805889070217,0.222043643392595);
#587=ELLIPSE('',#100578,0.239805704051158,0.22204316308686);
#588=ELLIPSE('',#100580,0.239805697269515,0.222042896630024);
#589=ELLIPSE('',#100581,0.239805882896034,0.222043378690203);
#590=ELLIPSE('',#100603,0.59937091393771,0.555630771250091);
#591=ELLIPSE('',#100604,0.599370291564638,0.555629413548847);
#592=ELLIPSE('',#100606,0.239805889068323,0.222043643388684);
#593=ELLIPSE('',#100607,0.239805704051787,0.222043163088177);
#594=ELLIPSE('',#100609,0.239805697269453,0.222042896629885);
#595=ELLIPSE('',#100610,0.239805882894651,0.222043378687309);
#596=ELLIPSE('',#100632,0.599370913937892,0.555630771250547);
#597=ELLIPSE('',#100633,0.599370291564007,0.555629413547481);
#598=ELLIPSE('',#100635,0.239805889068112,0.222043643388263);
#599=ELLIPSE('',#100636,0.2398057040517,0.222043163087922);
#600=ELLIPSE('',#100638,0.239805697267627,0.222042896626236);
#601=ELLIPSE('',#100639,0.239805882895515,0.222043378689114);
#602=ELLIPSE('',#100661,0.599370913937969,0.555630771250674);
#603=ELLIPSE('',#100662,0.599370291564076,0.555629413547814);
#604=ELLIPSE('',#100664,0.239805889070403,0.222043643392942);
#605=ELLIPSE('',#100665,0.239805704051981,0.222043163088492);
#606=ELLIPSE('',#100667,0.239805697268631,0.22204289662828);
#607=ELLIPSE('',#100668,0.239805882894013,0.222043378686015);
#608=ELLIPSE('',#100690,0.599370913938002,0.555630771250828);
#609=ELLIPSE('',#100691,0.599370291563501,0.555629413546602);
#610=ELLIPSE('',#100693,0.239805889069064,0.222043643390311);
#611=ELLIPSE('',#100694,0.239805704053694,0.222043163092107);
#612=ELLIPSE('',#100696,0.239805697269181,0.222042896629446);
#613=ELLIPSE('',#100697,0.239805882894764,0.22204337868757);
#614=ELLIPSE('',#100719,0.599370913937269,0.555630771249286);
#615=ELLIPSE('',#100720,0.599370291564187,0.555629413548004);
#616=ELLIPSE('',#100722,0.239805889070155,0.222043643392431);
#617=ELLIPSE('',#100723,0.239805704053049,0.222043163090734);
#618=ELLIPSE('',#100725,0.239805697269303,0.222042896629634);
#619=ELLIPSE('',#100726,0.239805882894004,0.222043378685988);
#620=ELLIPSE('',#100748,0.599370913936729,0.555630771248111);
#621=ELLIPSE('',#100749,0.599370291565056,0.555629413549728);
#622=ELLIPSE('',#100751,0.239805889071609,0.22204364339536);
#623=ELLIPSE('',#100752,0.239805704051184,0.222043163086902);
#624=ELLIPSE('',#100754,0.239805697269678,0.222042896630412);
#625=ELLIPSE('',#100755,0.239805882895219,0.222043378688562);
#626=ELLIPSE('',#100777,0.599370913936915,0.555630771248569);
#627=ELLIPSE('',#100778,0.599370291563785,0.555629413547203);
#628=ELLIPSE('',#100780,0.239805889069398,0.222043643390908);
#629=ELLIPSE('',#100781,0.239805704051609,0.22204316308779);
#630=ELLIPSE('',#100783,0.239805697268669,0.222042896628271);
#631=ELLIPSE('',#100784,0.239805882894659,0.222043378687315);
#632=ELLIPSE('',#100806,0.599370913939075,0.555630771253124);
#633=ELLIPSE('',#100807,0.599370291563701,0.555629413547064);
#634=ELLIPSE('',#100809,0.239805889070192,0.222043643392424);
#635=ELLIPSE('',#100810,0.239805704053763,0.222043163092232);
#636=ELLIPSE('',#100812,0.239805697270319,0.222042896631767);
#637=ELLIPSE('',#100813,0.239805882896116,0.222043378690362);
#638=ELLIPSE('',#100835,0.599370913937333,0.555630771249332);
#639=ELLIPSE('',#100836,0.599370291564169,0.555629413548037);
#640=ELLIPSE('',#100838,0.239805889068326,0.222043643388653);
#641=ELLIPSE('',#100839,0.2398057040546,0.222043163093935);
#642=ELLIPSE('',#100841,0.239805697269039,0.222042896629057);
#643=ELLIPSE('',#100842,0.239805882895526,0.222043378689145);
#644=ELLIPSE('',#100864,0.599370913937793,0.555630771250455);
#645=ELLIPSE('',#100865,0.599370291564337,0.555629413548237);
#646=ELLIPSE('',#100867,0.239805889070937,0.222043643394056);
#647=ELLIPSE('',#100868,0.239805704052185,0.222043163089078);
#648=ELLIPSE('',#100870,0.239805697268221,0.222042896627553);
#649=ELLIPSE('',#100871,0.239805882894638,0.222043378687215);
#650=ELLIPSE('',#100893,0.599370913938291,0.555630771251308);
#651=ELLIPSE('',#100894,0.599370291564336,0.555629413548396);
#652=ELLIPSE('',#100896,0.239805889070951,0.222043643394117);
#653=ELLIPSE('',#100897,0.239805704052956,0.222043163090467);
#654=ELLIPSE('',#100899,0.239805697268216,0.222042896627409);
#655=ELLIPSE('',#100900,0.239805882895213,0.222043378688343);
#656=ELLIPSE('',#100922,0.5993709139375,0.555630771249788);
#657=ELLIPSE('',#100923,0.599370291564678,0.555629413548944);
#658=ELLIPSE('',#100925,0.239805889072709,0.222043643397697);
#659=ELLIPSE('',#100926,0.239805704051998,0.222043163088687);
#660=ELLIPSE('',#100928,0.239805697269515,0.222042896630098);
#661=ELLIPSE('',#100929,0.239805882895996,0.222043378690038);
#662=ELLIPSE('',#100951,0.599370913936987,0.555630771248767);
#663=ELLIPSE('',#100952,0.599370291562368,0.55562941354422);
#664=ELLIPSE('',#100954,0.239805889071445,0.222043643395052);
#665=ELLIPSE('',#100955,0.239805704051795,0.222043163088107);
#666=ELLIPSE('',#100957,0.239805697270211,0.222042896631472);
#667=ELLIPSE('',#100958,0.239805882896537,0.222043378691172);
#668=ELLIPSE('',#100980,0.599370913937439,0.55563077124968);
#669=ELLIPSE('',#100981,0.599370291563737,0.555629413547156);
#670=ELLIPSE('',#100983,0.239805889069886,0.222043643391976);
#671=ELLIPSE('',#100984,0.23980570405216,0.222043163088966);
#672=ELLIPSE('',#100986,0.239805697271986,0.222042896635182);
#673=ELLIPSE('',#100987,0.239805882895563,0.222043378689248);
#674=ELLIPSE('',#101009,0.599370913935863,0.555630771246414);
#675=ELLIPSE('',#101010,0.599370291562441,0.555629413544446);
#676=ELLIPSE('',#101012,0.239805889069274,0.222043643390651);
#677=ELLIPSE('',#101013,0.239805704051074,0.222043163086558);
#678=ELLIPSE('',#101015,0.239805697268375,0.222042896627818);
#679=ELLIPSE('',#101016,0.239805882894152,0.222043378686232);
#680=ELLIPSE('',#101038,0.599370913938186,0.555630771251263);
#681=ELLIPSE('',#101039,0.599370291564916,0.555629413549503);
#682=ELLIPSE('',#101041,0.239805889069667,0.222043643391434);
#683=ELLIPSE('',#101042,0.239805704053102,0.222043163090824);
#684=ELLIPSE('',#101044,0.239805697269289,0.222042896629566);
#685=ELLIPSE('',#101045,0.239805882895496,0.222043378689093);
#686=ELLIPSE('',#101067,0.599370913937337,0.555630771249432);
#687=ELLIPSE('',#101068,0.599370291563716,0.555629413547141);
#688=ELLIPSE('',#101070,0.239805889070521,0.222043643393123);
#689=ELLIPSE('',#101071,0.239805704052324,0.222043163089135);
#690=ELLIPSE('',#101073,0.23980569726921,0.222042896629472);
#691=ELLIPSE('',#101074,0.239805882895584,0.222043378689238);
#692=ELLIPSE('',#101099,0.599370913936554,0.555630771247927);
#693=ELLIPSE('',#101100,0.599370291563314,0.55562941354626);
#694=ELLIPSE('',#101102,0.239805889071973,0.222043643396186);
#695=ELLIPSE('',#101103,0.239805704053213,0.222043163091114);
#696=ELLIPSE('',#101105,0.239805697271176,0.222042896633431);
#697=ELLIPSE('',#101106,0.239805882895932,0.222043378689924);
#698=ELLIPSE('',#101111,0.472049204510934,0.428376857312556);
#699=ELLIPSE('',#101112,0.472048618390948,0.428376332980169);
#700=ELLIPSE('',#101113,0.354420976867702,0.321488380363305);
#701=ELLIPSE('',#101114,0.35442112183661,0.321488565199684);
#702=ELLIPSE('',#101116,0.472048618673449,0.428376333587109);
#703=ELLIPSE('',#101117,0.472049204212692,0.428376856671643);
#704=ELLIPSE('',#101118,0.354421145892225,0.321488604125491);
#705=ELLIPSE('',#101119,0.354421089423447,0.321488612089807);
#706=ELLIPSE('',#101123,0.146692861887116,0.127051669379107);
#707=ELLIPSE('',#101135,0.146691465567175,0.127050784764067);
#708=ELLIPSE('',#101152,0.146692861887708,0.127051669379573);
#709=ELLIPSE('',#101163,0.146691465566821,0.12705078476379);
#710=ELLIPSE('',#101170,0.472049204509289,0.428376857309266);
#711=ELLIPSE('',#101171,0.472048618391431,0.428376332981064);
#712=ELLIPSE('',#101172,0.354420976861821,0.321488380351383);
#713=ELLIPSE('',#101173,0.35442112183555,0.321488565197576);
#714=ELLIPSE('',#101175,0.472048618673252,0.428376333586691);
#715=ELLIPSE('',#101176,0.472049204211803,0.42837685666992);
#716=ELLIPSE('',#101177,0.354421145892588,0.321488604126162);
#717=ELLIPSE('',#101178,0.354421089426214,0.321488612095312);
#718=ELLIPSE('',#101183,0.472049204510492,0.428376857311686);
#719=ELLIPSE('',#101184,0.472048618390858,0.428376332979975);
#720=ELLIPSE('',#101185,0.35442097686338,0.321488380354659);
#721=ELLIPSE('',#101186,0.354421121834003,0.321488565194468);
#722=ELLIPSE('',#101188,0.472048618674824,0.428376333589875);
#723=ELLIPSE('',#101189,0.472049204214783,0.428376856675792);
#724=ELLIPSE('',#101190,0.354421145894039,0.3214886041291);
#725=ELLIPSE('',#101191,0.354421089420356,0.321488612083628);
#726=ELLIPSE('',#101196,0.472049204512028,0.428376857314658);
#727=ELLIPSE('',#101197,0.472048618391491,0.428376332981219);
#728=ELLIPSE('',#101198,0.354420976864179,0.32148838035634);
#729=ELLIPSE('',#101199,0.354421121836554,0.321488565199535);
#730=ELLIPSE('',#101201,0.47204861867433,0.428376333588862);
#731=ELLIPSE('',#101202,0.472049204212632,0.428376856671534);
#732=ELLIPSE('',#101203,0.354421145892885,0.321488604126847);
#733=ELLIPSE('',#101204,0.354421089422622,0.32148861208819);
#734=ELLIPSE('',#101209,0.472049204510256,0.428376857311203);
#735=ELLIPSE('',#101210,0.472048618390729,0.428376332979685);
#736=ELLIPSE('',#101211,0.354420976865746,0.321488380359374);
#737=ELLIPSE('',#101212,0.354421121834367,0.321488565195157);
#738=ELLIPSE('',#101214,0.472048618674276,0.428376333588791);
#739=ELLIPSE('',#101215,0.47204920421503,0.428376856676324);
#740=ELLIPSE('',#101216,0.354421145892976,0.321488604126937);
#741=ELLIPSE('',#101217,0.354421089421022,0.321488612084937);
#742=ELLIPSE('',#101222,0.472049204511253,0.428376857313146);
#743=ELLIPSE('',#101223,0.472048618391128,0.428376332980535);
#744=ELLIPSE('',#101224,0.354420976867073,0.321488380362121);
#745=ELLIPSE('',#101225,0.354421121836193,0.321488565198845);
#746=ELLIPSE('',#101227,0.472048618674679,0.428376333589555);
#747=ELLIPSE('',#101228,0.472049204213367,0.428376856673016);
#748=ELLIPSE('',#101229,0.354421145894509,0.321488604130019);
#749=ELLIPSE('',#101230,0.354421089422398,0.321488612087834);
#750=ELLIPSE('',#101235,0.472049204510515,0.428376857311735);
#751=ELLIPSE('',#101236,0.472048618392408,0.428376332983092);
#752=ELLIPSE('',#101237,0.354420976869297,0.321488380366511);
#753=ELLIPSE('',#101238,0.354421121835321,0.321488565197107);
#754=ELLIPSE('',#101240,0.472048618673807,0.428376333587843);
#755=ELLIPSE('',#101241,0.472049204212756,0.428376856671762);
#756=ELLIPSE('',#101242,0.35442114589341,0.321488604127871);
#757=ELLIPSE('',#101243,0.354421089425903,0.321488612094688);
#758=ELLIPSE('',#101248,0.47204920451107,0.428376857312822);
#759=ELLIPSE('',#101249,0.472048618392803,0.42837633298386);
#760=ELLIPSE('',#101250,0.354420976860346,0.321488380348543);
#761=ELLIPSE('',#101251,0.354421121835633,0.321488565197806);
#762=ELLIPSE('',#101253,0.472048618674335,0.428376333588864);
#763=ELLIPSE('',#101254,0.472049204215952,0.428376856678111);
#764=ELLIPSE('',#101255,0.354421145892473,0.32148860412602);
#765=ELLIPSE('',#101256,0.354421089425772,0.321488612094473);
#766=ELLIPSE('',#101261,0.472049204509577,0.428376857309888);
#767=ELLIPSE('',#101262,0.47204861839227,0.428376332982796);
#768=ELLIPSE('',#101263,0.354420976869843,0.321488380367727);
#769=ELLIPSE('',#101264,0.354421121834772,0.321488565196016);
#770=ELLIPSE('',#101266,0.47204861867332,0.428376333586849);
#771=ELLIPSE('',#101267,0.472049204213765,0.428376856673737);
#772=ELLIPSE('',#101268,0.354421145891297,0.321488604123706);
#773=ELLIPSE('',#101269,0.354421089426494,0.321488612095895);
#774=ELLIPSE('',#101274,0.472049204513559,0.428376857317697);
#775=ELLIPSE('',#101275,0.472048618390786,0.42837633297985);
#776=ELLIPSE('',#101276,0.354420976865086,0.321488380358123);
#777=ELLIPSE('',#101277,0.354421121835652,0.321488565197754);
#778=ELLIPSE('',#101279,0.472048618673356,0.428376333586975);
#779=ELLIPSE('',#101280,0.472049204213523,0.428376856673277);
#780=ELLIPSE('',#101281,0.354421145893169,0.321488604127372);
#781=ELLIPSE('',#101282,0.354421089422401,0.321488612087849);
#782=ELLIPSE('',#101287,0.472049204510991,0.42837685731263);
#783=ELLIPSE('',#101288,0.472048618392257,0.428376332982714);
#784=ELLIPSE('',#101289,0.354420976868145,0.321488380364194);
#785=ELLIPSE('',#101290,0.354421121839984,0.321488565206443);
#786=ELLIPSE('',#101292,0.472048618673911,0.42837633358801);
#787=ELLIPSE('',#101293,0.472049204212241,0.428376856670714);
#788=ELLIPSE('',#101294,0.354421145893723,0.321488604128517);
#789=ELLIPSE('',#101295,0.354421089425117,0.321488612093203);
#790=ELLIPSE('',#101300,0.472049204510948,0.428376857312567);
#791=ELLIPSE('',#101301,0.472048618392567,0.428376332983328);
#792=ELLIPSE('',#101302,0.354420976870575,0.32148838036909);
#793=ELLIPSE('',#101303,0.354421121835812,0.32148856519803);
#794=ELLIPSE('',#101305,0.472048618673876,0.428376333587938);
#795=ELLIPSE('',#101306,0.472049204212521,0.428376856671341);
#796=ELLIPSE('',#101307,0.35442114589272,0.321488604126533);
#797=ELLIPSE('',#101308,0.354421089422786,0.321488612088435);
#798=ELLIPSE('',#101313,0.472049204511237,0.428376857313125);
#799=ELLIPSE('',#101314,0.472048618391984,0.4283763329822);
#800=ELLIPSE('',#101315,0.354420976866854,0.321488380361489);
#801=ELLIPSE('',#101316,0.354421121834466,0.321488565195394);
#802=ELLIPSE('',#101318,0.47204861867381,0.428376333587779);
#803=ELLIPSE('',#101319,0.472049204212592,0.428376856671459);
#804=ELLIPSE('',#101320,0.354421145893299,0.321488604127691);
#805=ELLIPSE('',#101321,0.354421089420226,0.321488612083325);
#806=ELLIPSE('',#101326,0.47204920451174,0.428376857314134);
#807=ELLIPSE('',#101327,0.472048618391901,0.428376332982063);
#808=ELLIPSE('',#101328,0.354420976864801,0.32148838035758);
#809=ELLIPSE('',#101329,0.354421121835268,0.321488565197031);
#810=ELLIPSE('',#101331,0.472048618674594,0.428376333589358);
#811=ELLIPSE('',#101332,0.47204920421434,0.428376856675008);
#812=ELLIPSE('',#101333,0.354421145891958,0.321488604125045);
#813=ELLIPSE('',#101334,0.354421089422399,0.321488612087739);
#814=ELLIPSE('',#101339,0.472049204509969,0.428376857310649);
#815=ELLIPSE('',#101340,0.472048618393256,0.428376332984763);
#816=ELLIPSE('',#101341,0.354420976867452,0.321488380362875);
#817=ELLIPSE('',#101342,0.354421121834484,0.321488565195343);
#818=ELLIPSE('',#101344,0.472048618673314,0.428376333586792);
#819=ELLIPSE('',#101345,0.47204920421347,0.428376856673174);
#820=ELLIPSE('',#101346,0.35442114589289,0.321488604126797);
#821=ELLIPSE('',#101347,0.354421089422546,0.321488612087928);
#822=ELLIPSE('',#101352,0.472049204510775,0.42837685731223);
#823=ELLIPSE('',#101353,0.472048618391864,0.428376332982002);
#824=ELLIPSE('',#101354,0.354420976864984,0.321488380357738);
#825=ELLIPSE('',#101355,0.354421121837171,0.321488565200749);
#826=ELLIPSE('',#101357,0.472048618673496,0.428376333587201);
#827=ELLIPSE('',#101358,0.472049204213379,0.428376856673032);
#828=ELLIPSE('',#101359,0.354421145891953,0.321488604124905);
#829=ELLIPSE('',#101360,0.354421089421714,0.321488612086365);
#830=ELLIPSE('',#101365,0.47204920451033,0.428376857311353);
#831=ELLIPSE('',#101366,0.47204861839312,0.428376332984429);
#832=ELLIPSE('',#101367,0.35442097686122,0.321488380350427);
#833=ELLIPSE('',#101368,0.354421121834249,0.321488565194965);
#834=ELLIPSE('',#101370,0.472048618675574,0.42837633359129);
#835=ELLIPSE('',#101371,0.472049204211857,0.428376856669993);
#836=ELLIPSE('',#101372,0.354421145893558,0.321488604128205);
#837=ELLIPSE('',#101373,0.354421089424109,0.321488612091213);
#838=ELLIPSE('',#101378,0.472049204509653,0.428376857310002);
#839=ELLIPSE('',#101379,0.47204861839197,0.428376332982155);
#840=ELLIPSE('',#101380,0.354420976862621,0.321488380353224);
#841=ELLIPSE('',#101381,0.354421121835799,0.321488565198063);
#842=ELLIPSE('',#101383,0.472048618674322,0.428376333588805);
#843=ELLIPSE('',#101384,0.472049204212596,0.428376856671498);
#844=ELLIPSE('',#101385,0.354421145890905,0.321488604122786);
#845=ELLIPSE('',#101386,0.354421089421594,0.321488612086012);
#846=ELLIPSE('',#101391,0.472049204510696,0.428376857312045);
#847=ELLIPSE('',#101392,0.472048618392718,0.428376332983668);
#848=ELLIPSE('',#101393,0.354420976864736,0.321488380357433);
#849=ELLIPSE('',#101394,0.3544211218364,0.321488565199259);
#850=ELLIPSE('',#101396,0.472048618674399,0.428376333588995);
#851=ELLIPSE('',#101397,0.472049204215212,0.428376856676614);
#852=ELLIPSE('',#101398,0.354421145892403,0.321488604125829);
#853=ELLIPSE('',#101399,0.354421089423517,0.321488612090008);
#854=ELLIPSE('',#101404,0.472049204512178,0.428376857315023);
#855=ELLIPSE('',#101405,0.47204861839185,0.428376332981941);
#856=ELLIPSE('',#101406,0.354420976867694,0.321488380363225);
#857=ELLIPSE('',#101407,0.354421121836556,0.321488565199582);
#858=ELLIPSE('',#101409,0.472048618673223,0.428376333586608);
#859=ELLIPSE('',#101410,0.472049204212149,0.428376856670589);
#860=ELLIPSE('',#101411,0.35442114589271,0.321488604126449);
#861=ELLIPSE('',#101412,0.354421089422371,0.321488612087722);
#862=ELLIPSE('',#101417,0.472049204509814,0.428376857310301);
#863=ELLIPSE('',#101418,0.472048618390664,0.428376332979562);
#864=ELLIPSE('',#101419,0.354420976864669,0.321488380357242);
#865=ELLIPSE('',#101420,0.354421121834253,0.321488565194901);
#866=ELLIPSE('',#101422,0.472048618673726,0.428376333587664);
#867=ELLIPSE('',#101423,0.472049204213629,0.428376856673542);
#868=ELLIPSE('',#101424,0.354421145892419,0.321488604125935);
#869=ELLIPSE('',#101425,0.354421089422999,0.321488612088916);
#870=ELLIPSE('',#101430,0.472049204511287,0.428376857313303);
#871=ELLIPSE('',#101431,0.472048618393151,0.428376332984527);
#872=ELLIPSE('',#101432,0.354420976866975,0.32148838036195);
#873=ELLIPSE('',#101433,0.354421121832796,0.321488565191982);
#874=ELLIPSE('',#101435,0.472048618673619,0.428376333587397);
#875=ELLIPSE('',#101436,0.472049204212268,0.428376856670815);
#876=ELLIPSE('',#101437,0.35442114589314,0.321488604127281);
#877=ELLIPSE('',#101438,0.354421089424284,0.321488612091627);
#878=ELLIPSE('',#101443,0.472049204509935,0.428376857310618);
#879=ELLIPSE('',#101444,0.472048618393844,0.428376332985917);
#880=ELLIPSE('',#101445,0.354420976863435,0.321488380354774);
#881=ELLIPSE('',#101446,0.354421121833964,0.321488565194345);
#882=ELLIPSE('',#101448,0.472048618673275,0.428376333586788);
#883=ELLIPSE('',#101449,0.472049204212259,0.428376856670844);
#884=ELLIPSE('',#101450,0.354421145892702,0.321488604126391);
#885=ELLIPSE('',#101451,0.35442108942423,0.321488612091314);
#886=ELLIPSE('',#101456,0.472049204511814,0.428376857314329);
#887=ELLIPSE('',#101457,0.472048618393361,0.42837633298497);
#888=ELLIPSE('',#101458,0.354420976864889,0.321488380357681);
#889=ELLIPSE('',#101459,0.354421121832822,0.321488565192075);
#890=ELLIPSE('',#101461,0.472048618674648,0.428376333589447);
#891=ELLIPSE('',#101462,0.472049204213791,0.428376856673861);
#892=ELLIPSE('',#101463,0.354421145891276,0.321488604123623);
#893=ELLIPSE('',#101464,0.35442108942329,0.321488612089543);
#894=ELLIPSE('',#101469,0.472049204510388,0.428376857311443);
#895=ELLIPSE('',#101470,0.472048618394646,0.428376332987444);
#896=ELLIPSE('',#101471,0.354420976863241,0.321488380354416);
#897=ELLIPSE('',#101472,0.354421121835884,0.321488565198253);
#898=ELLIPSE('',#101474,0.472048618674055,0.428376333588331);
#899=ELLIPSE('',#101475,0.472049204214137,0.428376856674488);
#900=ELLIPSE('',#101476,0.354421145893446,0.321488604127902);
#901=ELLIPSE('',#101477,0.354421089423459,0.321488612089795);
#902=ELLIPSE('',#101482,0.472049204513525,0.428376857317664);
#903=ELLIPSE('',#101483,0.472048618392254,0.428376332982779);
#904=ELLIPSE('',#101484,0.354420976860599,0.321488380349097);
#905=ELLIPSE('',#101485,0.354421121836793,0.321488565199991);
#906=ELLIPSE('',#101487,0.472048618674402,0.428376333588992);
#907=ELLIPSE('',#101488,0.472049204211988,0.428376856670282);
#908=ELLIPSE('',#101489,0.354421145893076,0.321488604127166);
#909=ELLIPSE('',#101490,0.354421089420329,0.32148861208354);
#910=ELLIPSE('',#101495,0.47204920451197,0.42837685731465);
#911=ELLIPSE('',#101496,0.472048618392666,0.428376332983572);
#912=ELLIPSE('',#101497,0.354420976864991,0.321488380357901);
#913=ELLIPSE('',#101498,0.354421121835,0.321488565196478);
#914=ELLIPSE('',#101500,0.472048618673531,0.4283763335873);
#915=ELLIPSE('',#101501,0.472049204213755,0.42837685667382);
#916=ELLIPSE('',#101502,0.354421145893716,0.321488604128501);
#917=ELLIPSE('',#101503,0.354421089417468,0.3214886120778);
#918=ELLIPSE('',#101508,0.472049204511671,0.428376857313973);
#919=ELLIPSE('',#101509,0.472048618392204,0.428376332982662);
#920=ELLIPSE('',#101510,0.354420976865648,0.321488380359166);
#921=ELLIPSE('',#101511,0.354421121836227,0.321488565198991);
#922=ELLIPSE('',#101513,0.472048618673305,0.428376333586812);
#923=ELLIPSE('',#101514,0.472049204212258,0.428376856670813);
#924=ELLIPSE('',#101515,0.354421145893316,0.321488604127761);
#925=ELLIPSE('',#101516,0.354421089421102,0.321488612085023);
#926=ELLIPSE('',#101521,0.472049204511125,0.42837685731293);
#927=ELLIPSE('',#101522,0.472048618393819,0.428376332985859);
#928=ELLIPSE('',#101523,0.354420976867475,0.321488380362911);
#929=ELLIPSE('',#101524,0.354421121834505,0.321488565195489);
#930=ELLIPSE('',#101526,0.472048618672661,0.428376333585526);
#931=ELLIPSE('',#101527,0.4720492042127,0.428376856671722);
#932=ELLIPSE('',#101528,0.35442114589236,0.321488604125723);
#933=ELLIPSE('',#101529,0.354421089420201,0.321488612083387);
#934=ELLIPSE('',#101534,0.472049204510718,0.428376857312093);
#935=ELLIPSE('',#101535,0.472048618392984,0.428376332984173);
#936=ELLIPSE('',#101536,0.35442097686326,0.321488380354402);
#937=ELLIPSE('',#101537,0.354421121836511,0.321488565199487);
#938=ELLIPSE('',#101539,0.472048618673284,0.428376333586807);
#939=ELLIPSE('',#101540,0.47204920421238,0.428376856671024);
#940=ELLIPSE('',#101541,0.354421145894016,0.32148860412904);
#941=ELLIPSE('',#101542,0.354421089421678,0.321488612086348);
#942=ELLIPSE('',#101545,0.472049204512392,0.428376857315418);
#943=ELLIPSE('',#101546,0.472048618392041,0.428376332982344);
#944=ELLIPSE('',#101547,0.354420976863591,0.321488380355001);
#945=ELLIPSE('',#101548,0.354421121837232,0.321488565200917);
#946=ELLIPSE('',#101550,0.472048618674192,0.428376333588603);
#947=ELLIPSE('',#101551,0.472049204214532,0.428376856675342);
#948=ELLIPSE('',#101552,0.354421145894906,0.32148860413083);
#949=ELLIPSE('',#101553,0.354421089421235,0.321488612085373);
#950=ELLIPSE('',#101558,0.472049204511627,0.428376857313931);
#951=ELLIPSE('',#101559,0.472048618392463,0.428376332983136);
#952=ELLIPSE('',#101560,0.3544209768649,0.321488380357729);
#953=ELLIPSE('',#101561,0.354421121832693,0.321488565191817);
#954=ELLIPSE('',#101563,0.472048618673316,0.428376333586818);
#955=ELLIPSE('',#101564,0.472049204211302,0.428376856668882);
#956=ELLIPSE('',#101565,0.354421145891833,0.321488604124742);
#957=ELLIPSE('',#101566,0.354421089425509,0.321488612093896);
#958=ELLIPSE('',#101571,0.472049204512195,0.428376857315009);
#959=ELLIPSE('',#101572,0.472048618391479,0.428376332981225);
#960=ELLIPSE('',#101573,0.354420976869266,0.321488380366468);
#961=ELLIPSE('',#101574,0.354421121835294,0.321488565196967);
#962=ELLIPSE('',#101576,0.47204861867312,0.428376333586429);
#963=ELLIPSE('',#101577,0.472049204214062,0.428376856674387);
#964=ELLIPSE('',#101578,0.354421145892696,0.321488604126356);
#965=ELLIPSE('',#101579,0.354421089419382,0.321488612081602);
#966=ELLIPSE('',#101584,0.472049204513345,0.428376857317346);
#967=ELLIPSE('',#101585,0.472048618392493,0.428376332983225);
#968=ELLIPSE('',#101586,0.354420976866613,0.321488380361188);
#969=ELLIPSE('',#101587,0.35442112183346,0.321488565193417);
#970=ELLIPSE('',#101589,0.472048618674328,0.428376333588841);
#971=ELLIPSE('',#101590,0.472049204213543,0.428376856673368);
#972=ELLIPSE('',#101591,0.354421145891292,0.321488604123538);
#973=ELLIPSE('',#101592,0.354421089420917,0.321488612084688);
#974=ELLIPSE('',#101597,0.472049204510815,0.42837685731222);
#975=ELLIPSE('',#101598,0.472048618394316,0.428376332986803);
#976=ELLIPSE('',#101599,0.354420976863249,0.321488380354374);
#977=ELLIPSE('',#101600,0.354421121838533,0.321488565203565);
#978=ELLIPSE('',#101602,0.47204861867473,0.428376333589591);
#979=ELLIPSE('',#101603,0.47204920421248,0.428376856671206);
#980=ELLIPSE('',#101604,0.354421145892991,0.321488604127081);
#981=ELLIPSE('',#101605,0.354421089424507,0.321488612091936);
#982=ELLIPSE('',#101610,0.472049204513034,0.428376857316677);
#983=ELLIPSE('',#101611,0.472048618393481,0.428376332985152);
#984=ELLIPSE('',#101612,0.354420976863262,0.321488380354344);
#985=ELLIPSE('',#101613,0.354421121836168,0.321488565198842);
#986=ELLIPSE('',#101615,0.472048618674509,0.428376333589219);
#987=ELLIPSE('',#101616,0.472049204212553,0.428376856671371);
#988=ELLIPSE('',#101617,0.354421145893113,0.321488604127279);
#989=ELLIPSE('',#101618,0.354421089422416,0.321488612087729);
#990=ELLIPSE('',#101623,0.472049204514185,0.42837685731902);
#991=ELLIPSE('',#101624,0.47204861839253,0.428376332983218);
#992=ELLIPSE('',#101625,0.354420976864303,0.321488380356576);
#993=ELLIPSE('',#101626,0.354421121838416,0.321488565203263);
#994=ELLIPSE('',#101628,0.472048618673455,0.428376333587087);
#995=ELLIPSE('',#101629,0.472049204213923,0.428376856674092);
#996=ELLIPSE('',#101630,0.354421145891633,0.321488604124298);
#997=ELLIPSE('',#101631,0.35442108941833,0.321488612079527);
#998=ELLIPSE('',#101636,0.472049204511433,0.428376857313588);
#999=ELLIPSE('',#101637,0.472048618392048,0.428376332982336);
#1000=ELLIPSE('',#101638,0.354420976865362,0.321488380358623);
#1001=ELLIPSE('',#101639,0.354421121836458,0.321488565199375);
#1002=ELLIPSE('',#101641,0.472048618673689,0.428376333587614);
#1003=ELLIPSE('',#101642,0.472049204215152,0.428376856676502);
#1004=ELLIPSE('',#101643,0.354421145892952,0.321488604126922);
#1005=ELLIPSE('',#101644,0.354421089419767,0.321488612082466);
#1006=ELLIPSE('',#101649,0.472049204510861,0.428376857312365);
#1007=ELLIPSE('',#101650,0.472048618392299,0.428376332982868);
#1008=ELLIPSE('',#101651,0.354420976866964,0.321488380361803);
#1009=ELLIPSE('',#101652,0.354421121832281,0.321488565191073);
#1010=ELLIPSE('',#101654,0.472048618674435,0.428376333589046);
#1011=ELLIPSE('',#101655,0.472049204214429,0.428376856675097);
#1012=ELLIPSE('',#101656,0.354421145893817,0.321488604128667);
#1013=ELLIPSE('',#101657,0.354421089421098,0.321488612084989);
#1014=ELLIPSE('',#101662,0.472049204511699,0.428376857314077);
#1015=ELLIPSE('',#101663,0.472048618391712,0.428376332981672);
#1016=ELLIPSE('',#101664,0.354420976866376,0.3214883803606);
#1017=ELLIPSE('',#101665,0.354421121836721,0.321488565199902);
#1018=ELLIPSE('',#101667,0.472048618673185,0.428376333586588);
#1019=ELLIPSE('',#101668,0.47204920421276,0.428376856671811);
#1020=ELLIPSE('',#101669,0.354421145893024,0.321488604127051);
#1021=ELLIPSE('',#101670,0.354421089423307,0.321488612089635);
#1022=ELLIPSE('',#101675,0.472049204511707,0.428376857314097);
#1023=ELLIPSE('',#101676,0.472048618390853,0.428376332979992);
#1024=ELLIPSE('',#101677,0.354420976863852,0.321488380355569);
#1025=ELLIPSE('',#101678,0.354421121835684,0.321488565197847);
#1026=ELLIPSE('',#101680,0.472048618673115,0.428376333586399);
#1027=ELLIPSE('',#101681,0.472049204211315,0.428376856668929);
#1028=ELLIPSE('',#101682,0.354421145892319,0.321488604125627);
#1029=ELLIPSE('',#101683,0.354421089421244,0.321488612085423);
#1030=ELLIPSE('',#101688,0.472049204511408,0.428376857313473);
#1031=ELLIPSE('',#101689,0.472048618391248,0.428376332980779);
#1032=ELLIPSE('',#101690,0.354420976866618,0.321488380361027);
#1033=ELLIPSE('',#101691,0.354421121834844,0.321488565196103);
#1034=ELLIPSE('',#101693,0.472048618673682,0.428376333587622);
#1035=ELLIPSE('',#101694,0.472049204214136,0.428376856674501);
#1036=ELLIPSE('',#101695,0.354421145893116,0.321488604127322);
#1037=ELLIPSE('',#101696,0.354421089422313,0.321488612087442);
#1038=ELLIPSE('',#101701,0.472049204511621,0.428376857313938);
#1039=ELLIPSE('',#101702,0.472048618390109,0.428376332978471);
#1040=ELLIPSE('',#101703,0.354420976868012,0.321488380363899);
#1041=ELLIPSE('',#101704,0.354421121837676,0.321488565201838);
#1042=ELLIPSE('',#101706,0.47204861867375,0.428376333587659);
#1043=ELLIPSE('',#101707,0.472049204213172,0.428376856672594);
#1044=ELLIPSE('',#101708,0.354421145890316,0.321488604121659);
#1045=ELLIPSE('',#101709,0.354421089424265,0.321488612091441);
#1046=ELLIPSE('',#101714,0.472049204512371,0.42837685731542);
#1047=ELLIPSE('',#101715,0.47204861839267,0.428376332983581);
#1048=ELLIPSE('',#101716,0.35442097686673,0.321488380361359);
#1049=ELLIPSE('',#101717,0.354421121837488,0.321488565201474);
#1050=ELLIPSE('',#101719,0.472048618674121,0.428376333588414);
#1051=ELLIPSE('',#101720,0.472049204212625,0.428376856671558);
#1052=ELLIPSE('',#101721,0.354421145894598,0.321488604130197);
#1053=ELLIPSE('',#101722,0.354421089423111,0.321488612089106);
#1054=ELLIPSE('',#101727,0.47204920451016,0.42837685731105);
#1055=ELLIPSE('',#101728,0.472048618391775,0.428376332981819);
#1056=ELLIPSE('',#101729,0.354420976864999,0.321488380357909);
#1057=ELLIPSE('',#101730,0.354421121834633,0.321488565195725);
#1058=ELLIPSE('',#101732,0.472048618674818,0.428376333589819);
#1059=ELLIPSE('',#101733,0.472049204213572,0.428376856673319);
#1060=ELLIPSE('',#101734,0.354421145892993,0.321488604126976);
#1061=ELLIPSE('',#101735,0.354421089423447,0.321488612089824);
#1062=ELLIPSE('',#101738,0.472049204509326,0.428376857309374);
#1063=ELLIPSE('',#101739,0.472048618392612,0.428376332983476);
#1064=ELLIPSE('',#101740,0.354420976864962,0.321488380357948);
#1065=ELLIPSE('',#101741,0.354421121838444,0.321488565203383);
#1066=ELLIPSE('',#101743,0.472048618673401,0.42837633358704);
#1067=ELLIPSE('',#101744,0.472049204213379,0.428376856673032);
#1068=ELLIPSE('',#101745,0.354421145892966,0.32148860412693);
#1069=ELLIPSE('',#101746,0.354421089421848,0.321488612086605);
#1070=ELLIPSE('',#101751,0.472049204510816,0.428376857312366);
#1071=ELLIPSE('',#101752,0.472048618391678,0.428376332981601);
#1072=ELLIPSE('',#101753,0.354420976865417,0.321488380358783);
#1073=ELLIPSE('',#101754,0.354421121835397,0.321488565197237);
#1074=ELLIPSE('',#101756,0.47204861867394,0.428376333588068);
#1075=ELLIPSE('',#101757,0.47204920421229,0.428376856670855);
#1076=ELLIPSE('',#101758,0.354421145891317,0.321488604123643);
#1077=ELLIPSE('',#101759,0.35442108941965,0.321488612082172);
#1078=ELLIPSE('',#101764,0.472049204509708,0.428376857310086);
#1079=ELLIPSE('',#101765,0.472048618392543,0.428376332983298);
#1080=ELLIPSE('',#101766,0.354420976862898,0.321488380353674);
#1081=ELLIPSE('',#101767,0.354421121837047,0.321488565200586);
#1082=ELLIPSE('',#101769,0.472048618674403,0.428376333589021);
#1083=ELLIPSE('',#101770,0.472049204212828,0.428376856671933);
#1084=ELLIPSE('',#101771,0.354421145890464,0.321488604121916);
#1085=ELLIPSE('',#101772,0.354421089425979,0.321488612094869);
#1086=ELLIPSE('',#101777,0.472049204511167,0.428376857313033);
#1087=ELLIPSE('',#101778,0.472048618392917,0.428376332984035);
#1088=ELLIPSE('',#101779,0.354420976866564,0.321488380361024);
#1089=ELLIPSE('',#101780,0.354421121837239,0.321488565201024);
#1090=ELLIPSE('',#101782,0.47204861867434,0.428376333588864);
#1091=ELLIPSE('',#101783,0.472049204215799,0.428376856677852);
#1092=ELLIPSE('',#101784,0.354421145893017,0.321488604127082);
#1093=ELLIPSE('',#101785,0.354421089422275,0.32148861208739);
#1094=ELLIPSE('',#101790,0.472049204510112,0.428376857310949);
#1095=ELLIPSE('',#101791,0.472048618392829,0.428376332983904);
#1096=ELLIPSE('',#101792,0.354420976868174,0.321488380364233);
#1097=ELLIPSE('',#101793,0.354421121835105,0.321488565196644);
#1098=ELLIPSE('',#101795,0.47204861867308,0.428376333586349);
#1099=ELLIPSE('',#101796,0.472049204212913,0.428376856672089);
#1100=ELLIPSE('',#101797,0.354421145893018,0.321488604127051);
#1101=ELLIPSE('',#101798,0.354421089419571,0.321488612081999);
#1102=ELLIPSE('',#101803,0.47204920451173,0.428376857314131);
#1103=ELLIPSE('',#101804,0.472048618391224,0.428376332980738);
#1104=ELLIPSE('',#101805,0.354420976867017,0.321488380361812);
#1105=ELLIPSE('',#101806,0.354421121834112,0.32148856519467);
#1106=ELLIPSE('',#101808,0.472048618673977,0.428376333588137);
#1107=ELLIPSE('',#101809,0.472049204213291,0.428376856672807);
#1108=ELLIPSE('',#101810,0.354421145890671,0.321488604122366);
#1109=ELLIPSE('',#101811,0.354421089422301,0.32148861208759);
#1110=ELLIPSE('',#101816,0.472049204510848,0.428376857312395);
#1111=ELLIPSE('',#101817,0.472048618392992,0.428376332984159);
#1112=ELLIPSE('',#101818,0.354420976860473,0.321488380348803);
#1113=ELLIPSE('',#101819,0.354421121834424,0.321488565195281);
#1114=ELLIPSE('',#101821,0.472048618672387,0.428376333584996);
#1115=ELLIPSE('',#101822,0.472049204212593,0.428376856671442);
#1116=ELLIPSE('',#101823,0.354421145892271,0.321488604125565);
#1117=ELLIPSE('',#101824,0.354421089420506,0.321488612083924);
#1118=ELLIPSE('',#101829,0.472049204511836,0.428376857314351);
#1119=ELLIPSE('',#101830,0.472048618392818,0.4283763329839);
#1120=ELLIPSE('',#101831,0.354420976866767,0.32148838036158);
#1121=ELLIPSE('',#101832,0.354421121834996,0.321488565196547);
#1122=ELLIPSE('',#101834,0.472048618675398,0.428376333590942);
#1123=ELLIPSE('',#101835,0.472049204211585,0.428376856669487);
#1124=ELLIPSE('',#101836,0.354421145891481,0.321488604124059);
#1125=ELLIPSE('',#101837,0.354421089423297,0.321488612089601);
#1126=ELLIPSE('',#101842,0.47204920451136,0.428376857313437);
#1127=ELLIPSE('',#101843,0.472048618391754,0.428376332981795);
#1128=ELLIPSE('',#101844,0.35442097686543,0.321488380358688);
#1129=ELLIPSE('',#101845,0.354421121834514,0.321488565195397);
#1130=ELLIPSE('',#101847,0.472048618674643,0.42837633358945);
#1131=ELLIPSE('',#101848,0.472049204212558,0.428376856671375);
#1132=ELLIPSE('',#101849,0.354421145894868,0.321488604130772);
#1133=ELLIPSE('',#101850,0.354421089425284,0.321488612093512);
#1134=ELLIPSE('',#101855,0.472049204512137,0.428376857314884);
#1135=ELLIPSE('',#101856,0.472048618392142,0.428376332982475);
#1136=ELLIPSE('',#101857,0.354420976863592,0.321488380355156);
#1137=ELLIPSE('',#101858,0.354421121836417,0.321488565199247);
#1138=ELLIPSE('',#101860,0.472048618672645,0.428376333585489);
#1139=ELLIPSE('',#101861,0.472049204214127,0.428376856674531);
#1140=ELLIPSE('',#101862,0.354421145892333,0.321488604125701);
#1141=ELLIPSE('',#101863,0.354421089418798,0.321488612080517);
#1142=ELLIPSE('',#101868,0.472049204508436,0.428376857307603);
#1143=ELLIPSE('',#101869,0.472048618391932,0.428376332982128);
#1144=ELLIPSE('',#101870,0.354420976866755,0.321488380361313);
#1145=ELLIPSE('',#101871,0.35442112183523,0.321488565196882);
#1146=ELLIPSE('',#101873,0.472048618675024,0.428376333590223);
#1147=ELLIPSE('',#101874,0.472049204210922,0.428376856668115);
#1148=ELLIPSE('',#101875,0.354421145894346,0.32148860412975);
#1149=ELLIPSE('',#101876,0.354421089422433,0.321488612087672);
#1150=ELLIPSE('',#101881,0.472049204511066,0.428376857312761);
#1151=ELLIPSE('',#101882,0.472048618392184,0.428376332982542);
#1152=ELLIPSE('',#101883,0.354420976862911,0.321488380353758);
#1153=ELLIPSE('',#101884,0.354421121836188,0.321488565198844);
#1154=ELLIPSE('',#101886,0.472048618673788,0.428376333587768);
#1155=ELLIPSE('',#101887,0.472049204212535,0.428376856671301);
#1156=ELLIPSE('',#101888,0.3544211458936,0.321488604128272);
#1157=ELLIPSE('',#101889,0.354421089422695,0.321488612088294);
#1158=ELLIPSE('',#101894,0.472049204512777,0.428376857316141);
#1159=ELLIPSE('',#101895,0.472048618393533,0.428376332985314);
#1160=ELLIPSE('',#101896,0.35442097686458,0.321488380357273);
#1161=ELLIPSE('',#101897,0.354421121835712,0.321488565197931);
#1162=ELLIPSE('',#101899,0.472048618676399,0.428376333592959);
#1163=ELLIPSE('',#101900,0.472049204210939,0.428376856668195);
#1164=ELLIPSE('',#101901,0.354421145890564,0.321488604122185);
#1165=ELLIPSE('',#101902,0.35442108942679,0.321488612096456);
#1166=ELLIPSE('',#101907,0.472049204511024,0.428376857312705);
#1167=ELLIPSE('',#101908,0.472048618392565,0.428376332983383);
#1168=ELLIPSE('',#101909,0.354420976866851,0.321488380361658);
#1169=ELLIPSE('',#101910,0.3544211218354,0.321488565197227);
#1170=ELLIPSE('',#101912,0.472048618674338,0.428376333588867);
#1171=ELLIPSE('',#101913,0.472049204211911,0.428376856670035);
#1172=ELLIPSE('',#101914,0.354421145891812,0.32148860412464);
#1173=ELLIPSE('',#101915,0.354421089427689,0.321488612098307);
#1174=ELLIPSE('',#101920,0.472049204510186,0.428376857311083);
#1175=ELLIPSE('',#101921,0.472048618393607,0.428376332985412);
#1176=ELLIPSE('',#101922,0.354420976862319,0.321488380352444);
#1177=ELLIPSE('',#101923,0.354421121836503,0.321488565199374);
#1178=ELLIPSE('',#101925,0.472048618672938,0.428376333586069);
#1179=ELLIPSE('',#101926,0.472049204213753,0.428376856673768);
#1180=ELLIPSE('',#101927,0.354421145891945,0.321488604124921);
#1181=ELLIPSE('',#101928,0.354421089420938,0.321488612084783);
#1182=ELLIPSE('',#102048,0.146692861885567,0.127051669378531);
#1183=ELLIPSE('',#102060,0.146691465567121,0.127050784764082);
#1184=ELLIPSE('',#102077,0.146692861887463,0.127051669378996);
#1185=ELLIPSE('',#102088,0.146691465567168,0.12705078476413);
#1186=ELLIPSE('',#102092,0.146692861888896,0.127051669380489);
#1187=ELLIPSE('',#102104,0.146691465567147,0.127050784764154);
#1188=ELLIPSE('',#102121,0.146692861886083,0.127051669378904);
#1189=ELLIPSE('',#102132,0.146691465566885,0.127050784763844);
#1190=ELLIPSE('',#102136,0.14669286188763,0.127051669380222);
#1191=ELLIPSE('',#102148,0.146691465566526,0.127050784763542);
#1192=ELLIPSE('',#102165,0.146692861887613,0.127051669379494);
#1193=ELLIPSE('',#102176,0.146691465566883,0.127050784763874);
#1194=ELLIPSE('',#102180,0.146692861887666,0.127051669380264);
#1195=ELLIPSE('',#102192,0.14669146556646,0.127050784763503);
#1196=ELLIPSE('',#102209,0.146692861889141,0.127051669380783);
#1197=ELLIPSE('',#102220,0.146691465567298,0.127050784764247);
#1198=ELLIPSE('',#102224,0.146692861888368,0.127051669379501);
#1199=ELLIPSE('',#102236,0.146691465567334,0.127050784764234);
#1200=ELLIPSE('',#102253,0.146692861886808,0.12705166937917);
#1201=ELLIPSE('',#102264,0.146691465566578,0.127050784763566);
#1202=ELLIPSE('',#102268,0.146692861888158,0.12705166937956);
#1203=ELLIPSE('',#102280,0.146691465566373,0.127050784763473);
#1204=ELLIPSE('',#102297,0.146692861888516,0.127051669379843);
#1205=ELLIPSE('',#102308,0.146691465566914,0.127050784763955);
#1206=ELLIPSE('',#102312,0.146692861888309,0.127051669380947);
#1207=ELLIPSE('',#102324,0.146691465567861,0.127050784764697);
#1208=ELLIPSE('',#102341,0.146692861885721,0.12705166937859);
#1209=ELLIPSE('',#102352,0.146691465566683,0.127050784763667);
#1210=ELLIPSE('',#102356,0.146692861888495,0.127051669380134);
#1211=ELLIPSE('',#102368,0.146691465567092,0.127050784764018);
#1212=ELLIPSE('',#102385,0.146692861888546,0.127051669380193);
#1213=ELLIPSE('',#102396,0.146691465567027,0.127050784763971);
#1214=ELLIPSE('',#102400,0.146692861887502,0.127051669379823);
#1215=ELLIPSE('',#102412,0.146691465567408,0.127050784764332);
#1216=ELLIPSE('',#102429,0.14669286188688,0.12705166937983);
#1217=ELLIPSE('',#102440,0.146691465567052,0.127050784763936);
#1218=ELLIPSE('',#102444,0.146692861890649,0.12705166938136);
#1219=ELLIPSE('',#102456,0.146691465567283,0.127050784764214);
#1220=ELLIPSE('',#102473,0.14669286188667,0.127051669379132);
#1221=ELLIPSE('',#102484,0.146691465566737,0.127050784763775);
#1222=ELLIPSE('',#102488,0.146692861885645,0.127051669379056);
#1223=ELLIPSE('',#102500,0.146691465566775,0.127050784763843);
#1224=ELLIPSE('',#102517,0.146692861887981,0.127051669380469);
#1225=ELLIPSE('',#102528,0.146691465567127,0.127050784764071);
#1226=ELLIPSE('',#102532,0.14669286188498,0.127051669377859);
#1227=ELLIPSE('',#102544,0.146691465566808,0.12705078476382);
#1228=ELLIPSE('',#102561,0.146692861889004,0.127051669380733);
#1229=ELLIPSE('',#102572,0.146691465567489,0.127050784764374);
#1230=ELLIPSE('',#102576,0.146692861885976,0.127051669378296);
#1231=ELLIPSE('',#102588,0.146691465567608,0.127050784764498);
#1232=ELLIPSE('',#102605,0.146692861886447,0.127051669378633);
#1233=ELLIPSE('',#102616,0.146691465566876,0.127050784763821);
#1234=ELLIPSE('',#102620,0.146692861886796,0.127051669378311);
#1235=ELLIPSE('',#102632,0.146691465567447,0.127050784764411);
#1236=ELLIPSE('',#102649,0.146692861889843,0.127051669381439);
#1237=ELLIPSE('',#102660,0.146691465567239,0.127050784764164);
#1238=ELLIPSE('',#102664,0.146692861890044,0.127051669381479);
#1239=ELLIPSE('',#102676,0.146691465567008,0.127050784763937);
#1240=ELLIPSE('',#102693,0.146692861885891,0.127051669378644);
#1241=ELLIPSE('',#102704,0.146691465567079,0.127050784764031);
#1242=ELLIPSE('',#102708,0.146692861888645,0.127051669380685);
#1243=ELLIPSE('',#102720,0.146691465567215,0.127050784764091);
#1244=ELLIPSE('',#102737,0.14669286188768,0.127051669379306);
#1245=ELLIPSE('',#102748,0.1466914655671,0.127050784764053);
#1246=ELLIPSE('',#102752,0.14669286188937,0.127051669381317);
#1247=ELLIPSE('',#102764,0.146691465567315,0.127050784764199);
#1248=ELLIPSE('',#102781,0.146692861887002,0.12705166937927);
#1249=ELLIPSE('',#102792,0.14669146556677,0.127050784763695);
#1250=ELLIPSE('',#102796,0.146692861887507,0.127051669380439);
#1251=ELLIPSE('',#102808,0.146691465567352,0.127050784764268);
#1252=ELLIPSE('',#102825,0.146692861887076,0.12705166937942);
#1253=ELLIPSE('',#102836,0.146691465566914,0.127050784763854);
#1254=ELLIPSE('',#102840,0.146692861887194,0.127051669379424);
#1255=ELLIPSE('',#102852,0.14669146556758,0.127050784764477);
#1256=ELLIPSE('',#102869,0.146692861888878,0.127051669380784);
#1257=ELLIPSE('',#102880,0.146691465567144,0.127050784764121);
#1258=ELLIPSE('',#102884,0.146692861887721,0.12705166937974);
#1259=ELLIPSE('',#102896,0.146691465567568,0.127050784764376);
#1260=ELLIPSE('',#102913,0.14669286188805,0.12705166938014);
#1261=ELLIPSE('',#102924,0.146691465567017,0.127050784763977);
#1262=ELLIPSE('',#102928,0.14669286188764,0.127051669379003);
#1263=ELLIPSE('',#102940,0.146691465566713,0.127050784763719);
#1264=ELLIPSE('',#102957,0.146692861888337,0.127051669380451);
#1265=ELLIPSE('',#102968,0.146691465567126,0.127050784763968);
#1266=ELLIPSE('',#102972,0.146692861887168,0.127051669379855);
#1267=ELLIPSE('',#102984,0.146691465566658,0.127050784763777);
#1268=ELLIPSE('',#103001,0.146692861887582,0.12705166937951);
#1269=ELLIPSE('',#103012,0.146691465567075,0.127050784764051);
#1270=ELLIPSE('',#103016,0.146692861888137,0.127051669380366);
#1271=ELLIPSE('',#103028,0.146691465567644,0.127050784764539);
#1272=ELLIPSE('',#103045,0.14669286188819,0.127051669379585);
#1273=ELLIPSE('',#103056,0.146691465567195,0.127050784764162);
#1274=ELLIPSE('',#103060,0.146692861889408,0.127051669380712);
#1275=ELLIPSE('',#103072,0.146691465566922,0.127050784763894);
#1276=ELLIPSE('',#103089,0.146692861888037,0.127051669379771);
#1277=ELLIPSE('',#103100,0.14669146556638,0.127050784763349);
#1278=ELLIPSE('',#103104,0.146692861889155,0.127051669380763);
#1279=ELLIPSE('',#103116,0.14669146556706,0.12705078476401);
#1280=ELLIPSE('',#103133,0.146692861882926,0.127051669377485);
#1281=ELLIPSE('',#103144,0.146691465567588,0.127050784764391);
#1282=ELLIPSE('',#103148,0.146692861885302,0.127051669379186);
#1283=ELLIPSE('',#103160,0.14669146556641,0.127050784763393);
#1284=ELLIPSE('',#103177,0.146692861883317,0.127051669378118);
#1285=ELLIPSE('',#103188,0.14669146556702,0.12705078476395);
#1286=ELLIPSE('',#103192,0.146692861885936,0.127051669377782);
#1287=ELLIPSE('',#103204,0.146691465567513,0.12705078476445);
#1288=ELLIPSE('',#103221,0.146692861888335,0.12705166938049);
#1289=ELLIPSE('',#103232,0.146691465567078,0.127050784763984);
#1290=ELLIPSE('',#103236,0.146692861887502,0.127051669379887);
#1291=ELLIPSE('',#103248,0.146691465567418,0.12705078476439);
#1292=ELLIPSE('',#103265,0.14669286188641,0.127051669379223);
#1293=ELLIPSE('',#103276,0.146691465568432,0.127050784765296);
#1294=ELLIPSE('',#103280,0.146692861886973,0.127051669378979);
#1295=ELLIPSE('',#103292,0.146691465567226,0.127050784764225);
#1296=ELLIPSE('',#103309,0.146692861887159,0.127051669379778);
#1297=ELLIPSE('',#103320,0.146691465566851,0.12705078476372);
#1298=ELLIPSE('',#103324,0.14669286188588,0.12705166937876);
#1299=ELLIPSE('',#103336,0.146691465567206,0.127050784764128);
#1300=ELLIPSE('',#103347,0.146692861889522,0.127051669380795);
#1301=ELLIPSE('',#103358,0.146691465567411,0.127050784764298);
#1302=ELLIPSE('',#103362,0.146692861889838,0.127051669381324);
#1303=ELLIPSE('',#103374,0.146691465567167,0.127050784764082);
#1304=ELLIPSE('',#103391,0.146692861887389,0.127051669379282);
#1305=ELLIPSE('',#103402,0.146691465566456,0.127050784763464);
#1306=ELLIPSE('',#103406,0.146692861889915,0.127051669381599);
#1307=ELLIPSE('',#103418,0.146691465567079,0.127050784764074);
#1308=ELLIPSE('',#103435,0.146692861886959,0.127051669379107);
#1309=ELLIPSE('',#103446,0.146691465565599,0.127050784762682);
#1310=ELLIPSE('',#103450,0.146692861886111,0.127051669378854);
#1311=ELLIPSE('',#103462,0.146691465566701,0.127050784763677);
#1312=ELLIPSE('',#103479,0.146692861887203,0.127051669379281);
#1313=ELLIPSE('',#103490,0.14669146556731,0.127050784764204);
#1314=ELLIPSE('',#103494,0.146692861883759,0.127051669378026);
#1315=ELLIPSE('',#103506,0.146691465567332,0.127050784764243);
#1316=ELLIPSE('',#103523,0.146692861886141,0.127051669379513);
#1317=ELLIPSE('',#103534,0.14669146556683,0.127050784763821);
#1318=ELLIPSE('',#103538,0.146692861885915,0.127051669378914);
#1319=ELLIPSE('',#103550,0.146691465566953,0.127050784763947);
#1320=ELLIPSE('',#103567,0.146692861888415,0.12705166938034);
#1321=ELLIPSE('',#103578,0.146691465567478,0.127050784764331);
#1322=ELLIPSE('',#103582,0.146692861891607,0.12705166938209);
#1323=ELLIPSE('',#103594,0.146691465566998,0.127050784763999);
#1324=ELLIPSE('',#103611,0.146692861888674,0.127051669380524);
#1325=ELLIPSE('',#103622,0.146691465567211,0.12705078476419);
#1326=ELLIPSE('',#103626,0.146692861883882,0.12705166937676);
#1327=ELLIPSE('',#103638,0.146691465566793,0.127050784763746);
#1328=ELLIPSE('',#103655,0.146692861887673,0.127051669380417);
#1329=ELLIPSE('',#103666,0.146691465567382,0.127050784764219);
#1330=ELLIPSE('',#103670,0.146692861887705,0.12705166937983);
#1331=ELLIPSE('',#103682,0.146691465566038,0.127050784763052);
#1332=ELLIPSE('',#103699,0.146692861889167,0.127051669380751);
#1333=ELLIPSE('',#103710,0.146691465567573,0.127050784764422);
#1334=ELLIPSE('',#103714,0.146692861889612,0.127051669381335);
#1335=ELLIPSE('',#103726,0.146691465567708,0.127050784764662);
#1336=ELLIPSE('',#103743,0.146692861889342,0.127051669380336);
#1337=ELLIPSE('',#103754,0.146691465567366,0.12705078476425);
#1338=ELLIPSE('',#103758,0.146692861886576,0.127051669378749);
#1339=ELLIPSE('',#103770,0.146691465566999,0.127050784763989);
#1340=ELLIPSE('',#103787,0.146692861884538,0.127051669377373);
#1341=ELLIPSE('',#103798,0.146691465567589,0.127050784764443);
#1342=ELLIPSE('',#103802,0.146692861890103,0.12705166938084);
#1343=ELLIPSE('',#103814,0.146691465567319,0.12705078476426);
#1344=ELLIPSE('',#103831,0.14669286189003,0.127051669381485);
#1345=ELLIPSE('',#103842,0.146691465567331,0.127050784764255);
#1346=ELLIPSE('',#103846,0.146692861888385,0.127051669380528);
#1347=ELLIPSE('',#103858,0.146691465566983,0.127050784763952);
#1348=ELLIPSE('',#103875,0.146692861884411,0.127051669377628);
#1349=ELLIPSE('',#103886,0.14669146556668,0.127050784763682);
#1350=ELLIPSE('',#103890,0.146692861886796,0.127051669378175);
#1351=ELLIPSE('',#103902,0.146691465566957,0.127050784763979);
#1352=ELLIPSE('',#103919,0.146692861887698,0.127051669379726);
#1353=ELLIPSE('',#103930,0.146691465567331,0.127050784764215);
#1354=ELLIPSE('',#103934,0.146692861885919,0.127051669378147);
#1355=ELLIPSE('',#103946,0.146691465566696,0.127050784763722);
#1356=ELLIPSE('',#103963,0.146692861886562,0.127051669379923);
#1357=ELLIPSE('',#103974,0.146691465567798,0.127050784764758);
#1358=ELLIPSE('',#103978,0.146692861888357,0.127051669380143);
#1359=ELLIPSE('',#103990,0.146691465567536,0.127050784764469);
#1360=ELLIPSE('',#104001,0.146692861886404,0.127051669379228);
#1361=ELLIPSE('',#104012,0.146691465567304,0.127050784764238);
#1362=ELLIPSE('',#104016,0.146692861888012,0.127051669380023);
#1363=ELLIPSE('',#104028,0.146691465567932,0.127050784764812);
#1364=ELLIPSE('',#104045,0.146692861885984,0.127051669378374);
#1365=ELLIPSE('',#104056,0.146691465567718,0.127050784764633);
#1366=ELLIPSE('',#104060,0.146692861888494,0.127051669381475);
#1367=ELLIPSE('',#104072,0.146691465566806,0.127050784763805);
#1368=ELLIPSE('',#104089,0.146692861886582,0.127051669379945);
#1369=ELLIPSE('',#104100,0.146691465566983,0.127050784763979);
#1370=ELLIPSE('',#104104,0.146692861885909,0.127051669378487);
#1371=ELLIPSE('',#104116,0.146691465566881,0.127050784763817);
#1372=ELLIPSE('',#104133,0.14669286188397,0.127051669377901);
#1373=ELLIPSE('',#104144,0.14669146556726,0.127050784764136);
#1374=ELLIPSE('',#104148,0.146692861885557,0.127051669377438);
#1375=ELLIPSE('',#104160,0.146691465567094,0.127050784764054);
#1376=ELLIPSE('',#104177,0.146692861888974,0.127051669380765);
#1377=ELLIPSE('',#104188,0.146691465567152,0.127050784764145);
#1378=ELLIPSE('',#104192,0.146692861888481,0.127051669380402);
#1379=ELLIPSE('',#104204,0.146691465566779,0.127050784763768);
#1380=ELLIPSE('',#104221,0.146692861888643,0.127051669380515);
#1381=ELLIPSE('',#104232,0.146691465567502,0.12705078476442);
#1382=ELLIPSE('',#104236,0.146692861890789,0.127051669381522);
#1383=ELLIPSE('',#104248,0.146691465566763,0.127050784763716);
#1384=ELLIPSE('',#104265,0.146692861888623,0.127051669380775);
#1385=ELLIPSE('',#104276,0.146691465566699,0.127050784763675);
#1386=ELLIPSE('',#104280,0.146692861888628,0.127051669380256);
#1387=ELLIPSE('',#104292,0.146691465566495,0.127050784763492);
#1388=ELLIPSE('',#104309,0.146692861887913,0.127051669380643);
#1389=ELLIPSE('',#104320,0.146691465568001,0.127050784764842);
#1390=ELLIPSE('',#104324,0.146692861885188,0.127051669378267);
#1391=ELLIPSE('',#104336,0.146691465566441,0.12705078476341);
#1392=ELLIPSE('',#104353,0.146692861887209,0.127051669379935);
#1393=ELLIPSE('',#104364,0.14669146556709,0.12705078476406);
#1394=ELLIPSE('',#104368,0.146692861890518,0.127051669381353);
#1395=ELLIPSE('',#104380,0.146691465567507,0.127050784764375);
#1396=ELLIPSE('',#104397,0.146692861883823,0.127051669377884);
#1397=ELLIPSE('',#104408,0.146691465567289,0.127050784764197);
#1398=ELLIPSE('',#104412,0.146692861890507,0.127051669381576);
#1399=ELLIPSE('',#104424,0.146691465567104,0.127050784764032);
#1400=ELLIPSE('',#104441,0.146692861883025,0.127051669377497);
#1401=ELLIPSE('',#104452,0.146691465567122,0.127050784764081);
#1402=ELLIPSE('',#104456,0.146692861888651,0.127051669380448);
#1403=ELLIPSE('',#104468,0.146691465567346,0.127050784764286);
#1404=ELLIPSE('',#104485,0.146692861886992,0.127051669380085);
#1405=ELLIPSE('',#104496,0.146691465566997,0.127050784763992);
#1406=ELLIPSE('',#104500,0.146692861887178,0.127051669379325);
#1407=ELLIPSE('',#104512,0.146691465567046,0.127050784763963);
#1408=ELLIPSE('',#104529,0.146692861888523,0.127051669381091);
#1409=ELLIPSE('',#104540,0.146691465567343,0.127050784764274);
#1410=ELLIPSE('',#104544,0.146692861885037,0.127051669378257);
#1411=ELLIPSE('',#104556,0.146691465567072,0.127050784763942);
#1412=ELLIPSE('',#104573,0.146692861888248,0.127051669380601);
#1413=ELLIPSE('',#104584,0.14669146556705,0.12705078476398);
#1414=ELLIPSE('',#104588,0.146692861886568,0.127051669378735);
#1415=ELLIPSE('',#104600,0.146691465566741,0.127050784763756);
#1416=ELLIPSE('',#104617,0.146692861887918,0.127051669379379);
#1417=ELLIPSE('',#104628,0.146691465566682,0.127050784763618);
#1418=ELLIPSE('',#104939,0.599370291563125,0.555629413545895);
#1419=ELLIPSE('',#104940,0.599370913936886,0.555630771248663);
#1420=ELLIPSE('',#104942,0.239805704053497,0.222043163091629);
#1421=ELLIPSE('',#104943,0.239805889070534,0.222043643393249);
#1422=ELLIPSE('',#104945,0.239805882896056,0.222043378690167);
#1423=ELLIPSE('',#104946,0.239805697268546,0.222042896628002);
#1424=ELLIPSE('',#104968,0.599370913936424,0.555630771247676);
#1425=ELLIPSE('',#104969,0.599370291563989,0.555629413547554);
#1426=ELLIPSE('',#104971,0.239805889069708,0.222043643391541);
#1427=ELLIPSE('',#104972,0.239805704051741,0.222043163087965);
#1428=ELLIPSE('',#104974,0.239805697269063,0.222042896629096);
#1429=ELLIPSE('',#104975,0.239805882896364,0.222043378690804);
#1430=ELLIPSE('',#104997,0.599370913938641,0.555630771252141);
#1431=ELLIPSE('',#104998,0.599370291563862,0.555629413547371);
#1432=ELLIPSE('',#105000,0.239805889070602,0.222043643393427);
#1433=ELLIPSE('',#105001,0.23980570405374,0.22204316309224);
#1434=ELLIPSE('',#105003,0.239805697270237,0.222042896631561);
#1435=ELLIPSE('',#105004,0.239805882896258,0.222043378690633);
#1436=ELLIPSE('',#105026,0.599370913937861,0.555630771250355);
#1437=ELLIPSE('',#105027,0.599370291563252,0.555629413546106);
#1438=ELLIPSE('',#105029,0.239805889071049,0.222043643394189);
#1439=ELLIPSE('',#105030,0.239805704053008,0.222043163090523);
#1440=ELLIPSE('',#105032,0.239805697269095,0.222042896629257);
#1441=ELLIPSE('',#105033,0.239805882896199,0.222043378690359);
#1442=ELLIPSE('',#105055,0.599370913937953,0.555630771250761);
#1443=ELLIPSE('',#105056,0.59937029156439,0.555629413548469);
#1444=ELLIPSE('',#105058,0.239805889069954,0.222043643392037);
#1445=ELLIPSE('',#105059,0.239805704051625,0.222043163087767);
#1446=ELLIPSE('',#105061,0.239805697269453,0.222042896629888);
#1447=ELLIPSE('',#105062,0.239805882894231,0.22204337868653);
#1448=ELLIPSE('',#105084,0.599370913935848,0.555630771246351);
#1449=ELLIPSE('',#105085,0.599370291563755,0.555629413547092);
#1450=ELLIPSE('',#105087,0.23980588907091,0.222043643394013);
#1451=ELLIPSE('',#105088,0.23980570405483,0.222043163094366);
#1452=ELLIPSE('',#105090,0.239805697270176,0.222042896631468);
#1453=ELLIPSE('',#105091,0.239805882895749,0.222043378689575);
#1454=ELLIPSE('',#105113,0.599370913938043,0.555630771251001);
#1455=ELLIPSE('',#105114,0.599370291563443,0.555629413546439);
#1456=ELLIPSE('',#105116,0.23980588907133,0.222043643394784);
#1457=ELLIPSE('',#105117,0.239805704053637,0.222043163091898);
#1458=ELLIPSE('',#105119,0.239805697268382,0.222042896627742);
#1459=ELLIPSE('',#105120,0.239805882894225,0.2220433786865);
#1460=ELLIPSE('',#105142,0.599370913937164,0.555630771249295);
#1461=ELLIPSE('',#105143,0.599370291564909,0.555629413549435);
#1462=ELLIPSE('',#105145,0.23980588907154,0.222043643395249);
#1463=ELLIPSE('',#105146,0.239805704053149,0.222043163090889);
#1464=ELLIPSE('',#105148,0.239805697270284,0.222042896631555);
#1465=ELLIPSE('',#105149,0.23980588289412,0.222043378686234);
#1466=ELLIPSE('',#105171,0.599370913937173,0.555630771249146);
#1467=ELLIPSE('',#105172,0.599370291561398,0.555629413542466);
#1468=ELLIPSE('',#105174,0.239805889070354,0.222043643392804);
#1469=ELLIPSE('',#105175,0.239805704053545,0.222043163091733);
#1470=ELLIPSE('',#105177,0.239805697271406,0.222042896633952);
#1471=ELLIPSE('',#105178,0.239805882895816,0.222043378689676);
#1472=ELLIPSE('',#105200,0.599370913937036,0.555630771248811);
#1473=ELLIPSE('',#105201,0.599370291563916,0.555629413547388);
#1474=ELLIPSE('',#105203,0.239805889071604,0.222043643395432);
#1475=ELLIPSE('',#105204,0.239805704053184,0.222043163090952);
#1476=ELLIPSE('',#105206,0.239805697268027,0.222042896626982);
#1477=ELLIPSE('',#105207,0.239805882895104,0.222043378688241);
#1478=ELLIPSE('',#105229,0.599370913938747,0.555630771252324);
#1479=ELLIPSE('',#105230,0.599370291563773,0.555629413547104);
#1480=ELLIPSE('',#105232,0.239805889069953,0.222043643391901);
#1481=ELLIPSE('',#105233,0.239805704053491,0.222043163091448);
#1482=ELLIPSE('',#105235,0.239805697268958,0.222042896628944);
#1483=ELLIPSE('',#105236,0.239805882896265,0.222043378690656);
#1484=ELLIPSE('',#105258,0.59937091393634,0.555630771247396);
#1485=ELLIPSE('',#105259,0.599370291564068,0.555629413547775);
#1486=ELLIPSE('',#105261,0.239805889068713,0.222043643389376);
#1487=ELLIPSE('',#105262,0.239805704053382,0.222043163091307);
#1488=ELLIPSE('',#105264,0.239805697270786,0.222042896632642);
#1489=ELLIPSE('',#105265,0.239805882894861,0.222043378687808);
#1490=ELLIPSE('',#105287,0.59937091393686,0.555630771248516);
#1491=ELLIPSE('',#105288,0.599370291565143,0.555629413549944);
#1492=ELLIPSE('',#105290,0.239805889071215,0.222043643394497);
#1493=ELLIPSE('',#105291,0.239805704050963,0.222043163086415);
#1494=ELLIPSE('',#105293,0.239805697269532,0.222042896630181);
#1495=ELLIPSE('',#105294,0.239805882893921,0.222043378685855);
#1496=ELLIPSE('',#105316,0.599370913938124,0.555630771251031);
#1497=ELLIPSE('',#105317,0.599370291563806,0.555629413547086);
#1498=ELLIPSE('',#105319,0.239805889070086,0.222043643392291);
#1499=ELLIPSE('',#105320,0.239805704054589,0.222043163093833);
#1500=ELLIPSE('',#105322,0.239805697267829,0.222042896626754);
#1501=ELLIPSE('',#105323,0.239805882895978,0.222043378689986);
#1502=ELLIPSE('',#105345,0.599370913938156,0.555630771251131);
#1503=ELLIPSE('',#105346,0.599370291565494,0.555629413550808);
#1504=ELLIPSE('',#105348,0.239805889069306,0.222043643390778);
#1505=ELLIPSE('',#105349,0.239805704052843,0.222043163090263);
#1506=ELLIPSE('',#105351,0.239805697267564,0.222042896626005);
#1507=ELLIPSE('',#105352,0.239805882895109,0.222043378688375);
#1508=ELLIPSE('',#105374,0.599370913936692,0.555630771248211);
#1509=ELLIPSE('',#105375,0.599370291564028,0.555629413547596);
#1510=ELLIPSE('',#105377,0.239805889070008,0.222043643392147);
#1511=ELLIPSE('',#105378,0.239805704053846,0.22204316309233);
#1512=ELLIPSE('',#105380,0.239805697267772,0.222042896626517);
#1513=ELLIPSE('',#105381,0.239805882894887,0.222043378687704);
#1514=ELLIPSE('',#105403,0.599370913937781,0.555630771250321);
#1515=ELLIPSE('',#105404,0.599370291564289,0.555629413548149);
#1516=ELLIPSE('',#105406,0.239805889071197,0.22204364339454);
#1517=ELLIPSE('',#105407,0.239805704052616,0.222043163089868);
#1518=ELLIPSE('',#105409,0.239805697268978,0.222042896629065);
#1519=ELLIPSE('',#105410,0.239805882893747,0.222043378685553);
#1520=ELLIPSE('',#105432,0.599370913937385,0.555630771249585);
#1521=ELLIPSE('',#105433,0.599370291563214,0.555629413545959);
#1522=ELLIPSE('',#105435,0.239805889069715,0.222043643391482);
#1523=ELLIPSE('',#105436,0.239805704052201,0.222043163088935);
#1524=ELLIPSE('',#105438,0.239805697268373,0.22204289662777);
#1525=ELLIPSE('',#105439,0.239805882895439,0.222043378688964);
#1526=ELLIPSE('',#105461,0.599370913937343,0.555630771249459);
#1527=ELLIPSE('',#105462,0.599370291565652,0.555629413550879);
#1528=ELLIPSE('',#105464,0.239805889069491,0.22204364339108);
#1529=ELLIPSE('',#105465,0.239805704052873,0.222043163090334);
#1530=ELLIPSE('',#105467,0.239805697269606,0.222042896630312);
#1531=ELLIPSE('',#105468,0.239805882895383,0.222043378688917);
#1532=ELLIPSE('',#105490,0.599370913936772,0.555630771248262);
#1533=ELLIPSE('',#105491,0.599370291561432,0.555629413542396);
#1534=ELLIPSE('',#105493,0.239805889069508,0.222043643391159);
#1535=ELLIPSE('',#105494,0.239805704052393,0.222043163089365);
#1536=ELLIPSE('',#105496,0.239805697268768,0.222042896628504);
#1537=ELLIPSE('',#105497,0.239805882896303,0.222043378690712);
#1538=ELLIPSE('',#105519,0.599370913936514,0.55563077124775);
#1539=ELLIPSE('',#105520,0.599370291562479,0.555629413544463);
#1540=ELLIPSE('',#105522,0.239805889069246,0.222043643390585);
#1541=ELLIPSE('',#105523,0.239805704052799,0.222043163090167);
#1542=ELLIPSE('',#105525,0.239805697269329,0.222042896629708);
#1543=ELLIPSE('',#105526,0.239805882896447,0.222043378691029);
#1544=ELLIPSE('',#105548,0.599370913936981,0.555630771248714);
#1545=ELLIPSE('',#105549,0.599370291561483,0.555629413542514);
#1546=ELLIPSE('',#105551,0.239805889069226,0.222043643390464);
#1547=ELLIPSE('',#105552,0.239805704052303,0.222043163089193);
#1548=ELLIPSE('',#105554,0.23980569726999,0.222042896631006);
#1549=ELLIPSE('',#105555,0.239805882894476,0.222043378686997);
#1550=ELLIPSE('',#105577,0.59937091393658,0.55563077124799);
#1551=ELLIPSE('',#105578,0.599370291562161,0.555629413543808);
#1552=ELLIPSE('',#105580,0.239805889071181,0.222043643394472);
#1553=ELLIPSE('',#105581,0.239805704051107,0.222043163086687);
#1554=ELLIPSE('',#105583,0.239805697269072,0.222042896629138);
#1555=ELLIPSE('',#105584,0.239805882893892,0.222043378685787);
#1556=ELLIPSE('',#105606,0.599370913936289,0.555630771247213);
#1557=ELLIPSE('',#105607,0.599370291564418,0.55562941354841);
#1558=ELLIPSE('',#105609,0.239805889069663,0.222043643391489);
#1559=ELLIPSE('',#105610,0.239805704053156,0.222043163090918);
#1560=ELLIPSE('',#105612,0.239805697269376,0.222042896629822);
#1561=ELLIPSE('',#105613,0.239805882896806,0.222043378691719);
#1562=ELLIPSE('',#105635,0.599370913938526,0.555630771252064);
#1563=ELLIPSE('',#105636,0.599370291563832,0.555629413547157);
#1564=ELLIPSE('',#105638,0.239805889069048,0.222043643390122);
#1565=ELLIPSE('',#105639,0.23980570405477,0.222043163094288);
#1566=ELLIPSE('',#105641,0.23980569726812,0.2220428966272);
#1567=ELLIPSE('',#105642,0.239805882894018,0.22204337868601);
#1568=ELLIPSE('',#105664,0.599370913936541,0.555630771247853);
#1569=ELLIPSE('',#105665,0.599370291564177,0.555629413547897);
#1570=ELLIPSE('',#105667,0.239805889069938,0.222043643391941);
#1571=ELLIPSE('',#105668,0.239805704053486,0.222043163091714);
#1572=ELLIPSE('',#105670,0.239805697268881,0.22204289662876);
#1573=ELLIPSE('',#105671,0.239805882895112,0.222043378688207);
#1574=ELLIPSE('',#105693,0.599370913938039,0.555630771250867);
#1575=ELLIPSE('',#105694,0.599370291564512,0.555629413548494);
#1576=ELLIPSE('',#105696,0.239805889069684,0.222043643391463);
#1577=ELLIPSE('',#105697,0.239805704053833,0.222043163092344);
#1578=ELLIPSE('',#105699,0.239805697268846,0.222042896628737);
#1579=ELLIPSE('',#105700,0.239805882897031,0.222043378692232);
#1580=ELLIPSE('',#105722,0.599370913936877,0.555630771248588);
#1581=ELLIPSE('',#105723,0.599370291562475,0.555629413544577);
#1582=ELLIPSE('',#105725,0.239805889068947,0.222043643389968);
#1583=ELLIPSE('',#105726,0.239805704052611,0.222043163089871);
#1584=ELLIPSE('',#105728,0.23980569726888,0.222042896628872);
#1585=ELLIPSE('',#105729,0.239805882896037,0.222043378690158);
#1586=ELLIPSE('',#105751,0.599370913936578,0.55563077124794);
#1587=ELLIPSE('',#105752,0.599370291564127,0.555629413547831);
#1588=ELLIPSE('',#105754,0.239805889069815,0.2220436433917);
#1589=ELLIPSE('',#105755,0.23980570405164,0.222043163087847);
#1590=ELLIPSE('',#105757,0.23980569726956,0.222042896630156);
#1591=ELLIPSE('',#105758,0.239805882895319,0.222043378688701);
#1592=ELLIPSE('',#105780,0.599370913938708,0.555630771252267);
#1593=ELLIPSE('',#105781,0.599370291563981,0.555629413547567);
#1594=ELLIPSE('',#105783,0.239805889070531,0.222043643393195);
#1595=ELLIPSE('',#105784,0.239805704052955,0.222043163090464);
#1596=ELLIPSE('',#105786,0.239805697267724,0.222042896626334);
#1597=ELLIPSE('',#105787,0.239805882894363,0.222043378686709);
#1598=ELLIPSE('',#105809,0.599370913938198,0.555630771251102);
#1599=ELLIPSE('',#105810,0.599370291564309,0.555629413548225);
#1600=ELLIPSE('',#105812,0.239805889069912,0.22204364339194);
#1601=ELLIPSE('',#105813,0.239805704052815,0.222043163090226);
#1602=ELLIPSE('',#105815,0.239805697269805,0.222042896630579);
#1603=ELLIPSE('',#105816,0.239805882895327,0.222043378688781);
#1604=ELLIPSE('',#105838,0.5993709139359,0.555630771246453);
#1605=ELLIPSE('',#105839,0.599370291564582,0.555629413548754);
#1606=ELLIPSE('',#105841,0.239805889071206,0.222043643394522);
#1607=ELLIPSE('',#105842,0.239805704053369,0.222043163091383);
#1608=ELLIPSE('',#105844,0.239805697269504,0.222042896630047);
#1609=ELLIPSE('',#105845,0.239805882894382,0.222043378686745);
#1610=ELLIPSE('',#105867,0.599370913938674,0.555630771252144);
#1611=ELLIPSE('',#105868,0.599370291562963,0.555629413545488);
#1612=ELLIPSE('',#105870,0.239805889069481,0.222043643391073);
#1613=ELLIPSE('',#105871,0.239805704050848,0.222043163086202);
#1614=ELLIPSE('',#105873,0.239805697268431,0.222042896627882);
#1615=ELLIPSE('',#105874,0.239805882896349,0.222043378690827);
#1616=ELLIPSE('',#105896,0.599370913936395,0.555630771247448);
#1617=ELLIPSE('',#105897,0.599370291566618,0.555629413552874);
#1618=ELLIPSE('',#105899,0.239805889069956,0.222043643391995);
#1619=ELLIPSE('',#105900,0.239805704052727,0.222043163090096);
#1620=ELLIPSE('',#105902,0.239805697269363,0.222042896629784);
#1621=ELLIPSE('',#105903,0.23980588289559,0.222043378689183);
#1622=ELLIPSE('',#105925,0.599370913937641,0.555630771249903);
#1623=ELLIPSE('',#105926,0.599370291564417,0.555629413548418);
#1624=ELLIPSE('',#105928,0.239805889070735,0.22204364339359);
#1625=ELLIPSE('',#105929,0.239805704054714,0.222043163094138);
#1626=ELLIPSE('',#105931,0.239805697269139,0.222042896629365);
#1627=ELLIPSE('',#105932,0.239805882894918,0.222043378687834);
#1628=ELLIPSE('',#105954,0.599370913937249,0.555630771249287);
#1629=ELLIPSE('',#105955,0.599370291563887,0.555629413547403);
#1630=ELLIPSE('',#105957,0.239805889070777,0.222043643393741);
#1631=ELLIPSE('',#105958,0.239805704051975,0.22204316308848);
#1632=ELLIPSE('',#105960,0.239805697266916,0.222042896624693);
#1633=ELLIPSE('',#105961,0.239805882895061,0.222043378688168);
#1634=ELLIPSE('',#105983,0.599370913938545,0.555630771251985);
#1635=ELLIPSE('',#105984,0.599370291562687,0.555629413544967);
#1636=ELLIPSE('',#105986,0.239805889070212,0.222043643392528);
#1637=ELLIPSE('',#105987,0.239805704051763,0.222043163088153);
#1638=ELLIPSE('',#105989,0.239805697268783,0.222042896628616);
#1639=ELLIPSE('',#105990,0.239805882896158,0.222043378690411);
#1640=ELLIPSE('',#106012,0.599370913937149,0.555630771249181);
#1641=ELLIPSE('',#106013,0.599370291564607,0.555629413548761);
#1642=ELLIPSE('',#106015,0.239805889070846,0.222043643393813);
#1643=ELLIPSE('',#106016,0.239805704053588,0.222043163091749);
#1644=ELLIPSE('',#106018,0.239805697268943,0.222042896628931);
#1645=ELLIPSE('',#106019,0.239805882894556,0.222043378687108);
#1646=ELLIPSE('',#106041,0.599370913936176,0.555630771247153);
#1647=ELLIPSE('',#106042,0.59937029156489,0.555629413549416);
#1648=ELLIPSE('',#106044,0.239805889070307,0.222043643392796);
#1649=ELLIPSE('',#106045,0.239805704052103,0.22204316308874);
#1650=ELLIPSE('',#106047,0.239805697269308,0.222042896629674);
#1651=ELLIPSE('',#106048,0.239805882894806,0.222043378687586);
#1652=ELLIPSE('',#106070,0.599370913937901,0.555630771250564);
#1653=ELLIPSE('',#106071,0.599370291564246,0.555629413548082);
#1654=ELLIPSE('',#106073,0.239805889069668,0.222043643391381);
#1655=ELLIPSE('',#106074,0.239805704051946,0.222043163088454);
#1656=ELLIPSE('',#106076,0.239805697269087,0.222042896629094);
#1657=ELLIPSE('',#106077,0.239805882896672,0.222043378691442);
#1658=ELLIPSE('',#106099,0.599370913936996,0.555630771248784);
#1659=ELLIPSE('',#106100,0.599370291563568,0.555629413546736);
#1660=ELLIPSE('',#106102,0.239805889067455,0.22204364338699);
#1661=ELLIPSE('',#106103,0.239805704051744,0.222043163088029);
#1662=ELLIPSE('',#106105,0.239805697267273,0.222042896625362);
#1663=ELLIPSE('',#106106,0.239805882896202,0.22204337869045);
#1664=ELLIPSE('',#106128,0.599370913939066,0.555630771253014);
#1665=ELLIPSE('',#106129,0.599370291562359,0.555629413544269);
#1666=ELLIPSE('',#106131,0.239805889070273,0.222043643392718);
#1667=ELLIPSE('',#106132,0.239805704052602,0.222043163089835);
#1668=ELLIPSE('',#106134,0.239805697269778,0.222042896630685);
#1669=ELLIPSE('',#106135,0.239805882895276,0.222043378688557);
#1670=ELLIPSE('',#106157,0.599370913937787,0.555630771250463);
#1671=ELLIPSE('',#106158,0.599370291563937,0.555629413547465);
#1672=ELLIPSE('',#106160,0.23980588907131,0.222043643394858);
#1673=ELLIPSE('',#106161,0.239805704051925,0.222043163088452);
#1674=ELLIPSE('',#106163,0.239805697266862,0.222042896624485);
#1675=ELLIPSE('',#106164,0.239805882895514,0.222043378689123);
#1676=ELLIPSE('',#106186,0.599370913938338,0.555630771251542);
#1677=ELLIPSE('',#106187,0.599370291563512,0.555629413546666);
#1678=ELLIPSE('',#106189,0.239805889068806,0.222043643389686);
#1679=ELLIPSE('',#106190,0.239805704052207,0.222043163089033);
#1680=ELLIPSE('',#106192,0.239805697271128,0.222042896633369);
#1681=ELLIPSE('',#106193,0.239805882895001,0.222043378688052);
#1682=ELLIPSE('',#106215,0.599370913937752,0.555630771250446);
#1683=ELLIPSE('',#106216,0.599370291564464,0.555629413548618);
#1684=ELLIPSE('',#106218,0.239805889071983,0.222043643396124);
#1685=ELLIPSE('',#106219,0.239805704051923,0.222043163088459);
#1686=ELLIPSE('',#106221,0.239805697268376,0.222042896627738);
#1687=ELLIPSE('',#106222,0.23980588289422,0.222043378686507);
#1688=ELLIPSE('',#106244,0.599370913937345,0.555630771249436);
#1689=ELLIPSE('',#106245,0.59937029156196,0.555629413543465);
#1690=ELLIPSE('',#106247,0.239805889069961,0.222043643392058);
#1691=ELLIPSE('',#106248,0.239805704053478,0.222043163091603);
#1692=ELLIPSE('',#106250,0.239805697269098,0.22204289662929);
#1693=ELLIPSE('',#106251,0.2398058828958,0.22204337868961);
#1694=ELLIPSE('',#106273,0.599370913937037,0.555630771248897);
#1695=ELLIPSE('',#106274,0.599370291562031,0.555629413543674);
#1696=ELLIPSE('',#106276,0.239805889069035,0.22204364339024);
#1697=ELLIPSE('',#106277,0.239805704052574,0.222043163089708);
#1698=ELLIPSE('',#106279,0.239805697269961,0.222042896631028);
#1699=ELLIPSE('',#106280,0.23980588289584,0.222043378689655);
#1700=ELLIPSE('',#106302,0.599370913936974,0.555630771248813);
#1701=ELLIPSE('',#106303,0.599370291564014,0.555629413547602);
#1702=ELLIPSE('',#106305,0.239805889071759,0.222043643395731);
#1703=ELLIPSE('',#106306,0.239805704052857,0.22204316309031);
#1704=ELLIPSE('',#106308,0.239805697268703,0.222042896628388);
#1705=ELLIPSE('',#106309,0.23980588289455,0.222043378687117);
#1706=ELLIPSE('',#106331,0.599370913936989,0.55563077124864);
#1707=ELLIPSE('',#106332,0.599370291565194,0.555629413549919);
#1708=ELLIPSE('',#106334,0.239805889070791,0.222043643393766);
#1709=ELLIPSE('',#106335,0.239805704052858,0.22204316309034);
#1710=ELLIPSE('',#106337,0.239805697267834,0.222042896626616);
#1711=ELLIPSE('',#106338,0.239805882894524,0.222043378687112);
#1712=ELLIPSE('',#106360,0.599370913937548,0.555630771249916);
#1713=ELLIPSE('',#106361,0.599370291564909,0.555629413549445);
#1714=ELLIPSE('',#106363,0.239805889070836,0.222043643393712);
#1715=ELLIPSE('',#106364,0.239805704052287,0.222043163089176);
#1716=ELLIPSE('',#106366,0.239805697267837,0.222042896626536);
#1717=ELLIPSE('',#106367,0.239805882896042,0.222043378690122);
#1718=ELLIPSE('',#106389,0.599370913937273,0.555630771249356);
#1719=ELLIPSE('',#106390,0.599370291565437,0.555629413550552);
#1720=ELLIPSE('',#106392,0.239805889070935,0.222043643394021);
#1721=ELLIPSE('',#106393,0.239805704053519,0.222043163091695);
#1722=ELLIPSE('',#106395,0.239805697270266,0.222042896631555);
#1723=ELLIPSE('',#106396,0.239805882895611,0.222043378689254);
#1724=ELLIPSE('',#106418,0.599370913937078,0.555630771248908);
#1725=ELLIPSE('',#106419,0.599370291563712,0.555629413547031);
#1726=ELLIPSE('',#106421,0.239805889071625,0.222043643395324);
#1727=ELLIPSE('',#106422,0.239805704053465,0.222043163091574);
#1728=ELLIPSE('',#106424,0.239805697270216,0.222042896631521);
#1729=ELLIPSE('',#106425,0.239805882894735,0.222043378687381);
#1730=ELLIPSE('',#106447,0.59937091393725,0.555630771249377);
#1731=ELLIPSE('',#106448,0.599370291564746,0.55562941354917);
#1732=ELLIPSE('',#106450,0.239805889070006,0.222043643392107);
#1733=ELLIPSE('',#106451,0.239805704052258,0.222043163089137);
#1734=ELLIPSE('',#106453,0.239805697270427,0.222042896631951);
#1735=ELLIPSE('',#106454,0.239805882895842,0.22204337868974);
#1736=ELLIPSE('',#106476,0.599370913936956,0.555630771248539);
#1737=ELLIPSE('',#106477,0.599370291565833,0.555629413551388);
#1738=ELLIPSE('',#106479,0.239805889069105,0.222043643390322);
#1739=ELLIPSE('',#106480,0.239805704054033,0.222043163092783);
#1740=ELLIPSE('',#106482,0.239805697268147,0.222042896627119);
#1741=ELLIPSE('',#106483,0.239805882895254,0.222043378688474);
#1742=ELLIPSE('',#106505,0.599370913937186,0.555630771249278);
#1743=ELLIPSE('',#106506,0.59937029156173,0.555629413543073);
#1744=ELLIPSE('',#106508,0.239805889070897,0.222043643393939);
#1745=ELLIPSE('',#106509,0.239805704052673,0.222043163089943);
#1746=ELLIPSE('',#106511,0.239805697269764,0.222042896630456);
#1747=ELLIPSE('',#106512,0.239805882895431,0.222043378688825);
#1748=ELLIPSE('',#106534,0.59937091393695,0.555630771248692);
#1749=ELLIPSE('',#106535,0.599370291563103,0.555629413545827);
#1750=ELLIPSE('',#106537,0.239805889069582,0.222043643391203);
#1751=ELLIPSE('',#106538,0.239805704053097,0.22204316309083);
#1752=ELLIPSE('',#106540,0.239805697270417,0.222042896631992);
#1753=ELLIPSE('',#106541,0.239805882894859,0.222043378687672);
#1754=ELLIPSE('',#106563,0.599370913936272,0.555630771247367);
#1755=ELLIPSE('',#106564,0.599370291562787,0.555629413545066);
#1756=ELLIPSE('',#106566,0.239805889069898,0.222043643391812);
#1757=ELLIPSE('',#106567,0.239805704053116,0.222043163090822);
#1758=ELLIPSE('',#106569,0.23980569727021,0.222042896631462);
#1759=ELLIPSE('',#106570,0.239805882896488,0.222043378691088);
#1760=ELLIPSE('',#106592,0.599370913937577,0.555630771249974);
#1761=ELLIPSE('',#106593,0.599370291563603,0.555629413546849);
#1762=ELLIPSE('',#106595,0.239805889069516,0.222043643391181);
#1763=ELLIPSE('',#106596,0.239805704052191,0.222043163088941);
#1764=ELLIPSE('',#106598,0.239805697269283,0.222042896629651);
#1765=ELLIPSE('',#106599,0.239805882895395,0.222043378688882);
#1766=ELLIPSE('',#106621,0.599370913936449,0.555630771247687);
#1767=ELLIPSE('',#106622,0.599370291564252,0.555629413548182);
#1768=ELLIPSE('',#106624,0.239805889069627,0.222043643391383);
#1769=ELLIPSE('',#106625,0.23980570405205,0.22204316308868);
#1770=ELLIPSE('',#106627,0.239805697270006,0.22204289663112);
#1771=ELLIPSE('',#106628,0.239805882895028,0.222043378688055);
#1772=ELLIPSE('',#106653,0.599370913935561,0.55563077124596);
#1773=ELLIPSE('',#106654,0.599370291562403,0.555629413544383);
#1774=ELLIPSE('',#106656,0.239805889070797,0.222043643393652);
#1775=ELLIPSE('',#106657,0.23980570405278,0.222043163090117);
#1776=ELLIPSE('',#106659,0.239805697267951,0.222042896626835);
#1777=ELLIPSE('',#106660,0.239805882896207,0.222043378690511);
#1778=ELLIPSE('',#106665,0.472049204511299,0.428376857313292);
#1779=ELLIPSE('',#106666,0.472048618391423,0.428376332981108);
#1780=ELLIPSE('',#106667,0.354420976864826,0.321488380357502);
#1781=ELLIPSE('',#106668,0.354421121835649,0.321488565197775);
#1782=ELLIPSE('',#106670,0.472048618673416,0.428376333587049);
#1783=ELLIPSE('',#106671,0.472049204213287,0.428376856672832);
#1784=ELLIPSE('',#106672,0.354421145892816,0.321488604126673);
#1785=ELLIPSE('',#106673,0.354421089423499,0.321488612089889);
#1786=ELLIPSE('',#106677,0.146692861887334,0.127051669379536);
#1787=ELLIPSE('',#106689,0.146691465566744,0.127050784763687);
#1788=ELLIPSE('',#106706,0.146692861887626,0.127051669379765);
#1789=ELLIPSE('',#106717,0.146691465566936,0.127050784763915);
#1790=ELLIPSE('',#106724,0.47204920451043,0.42837685731154);
#1791=ELLIPSE('',#106725,0.472048618392884,0.428376332983992);
#1792=ELLIPSE('',#106726,0.354420976864662,0.321488380357232);
#1793=ELLIPSE('',#106727,0.354421121835341,0.321488565197164);
#1794=ELLIPSE('',#106729,0.472048618673052,0.428376333586304);
#1795=ELLIPSE('',#106730,0.472049204212421,0.428376856671127);
#1796=ELLIPSE('',#106731,0.354421145893183,0.321488604127369);
#1797=ELLIPSE('',#106732,0.354421089422911,0.321488612088706);
#1798=ELLIPSE('',#106737,0.472049204511464,0.428376857313639);
#1799=ELLIPSE('',#106738,0.472048618392123,0.428376332982553);
#1800=ELLIPSE('',#106739,0.354420976865553,0.321488380358974);
#1801=ELLIPSE('',#106740,0.354421121835029,0.321488565196566);
#1802=ELLIPSE('',#106742,0.472048618673971,0.42837633358811);
#1803=ELLIPSE('',#106743,0.472049204213955,0.428376856674181);
#1804=ELLIPSE('',#106744,0.354421145892627,0.321488604126292);
#1805=ELLIPSE('',#106745,0.354421089421795,0.321488612086537);
#1806=ELLIPSE('',#106750,0.47204920451058,0.428376857311775);
#1807=ELLIPSE('',#106751,0.472048618391896,0.428376332982026);
#1808=ELLIPSE('',#106752,0.354420976864346,0.321488380356575);
#1809=ELLIPSE('',#106753,0.354421121837741,0.321488565201974);
#1810=ELLIPSE('',#106755,0.472048618673973,0.428376333588145);
#1811=ELLIPSE('',#106756,0.472049204212974,0.428376856672254);
#1812=ELLIPSE('',#106757,0.354421145894067,0.321488604129196);
#1813=ELLIPSE('',#106758,0.354421089421142,0.321488612085148);
#1814=ELLIPSE('',#106763,0.472049204511116,0.42837685731288);
#1815=ELLIPSE('',#106764,0.472048618392269,0.428376332982734);
#1816=ELLIPSE('',#106765,0.354420976863336,0.321488380354612);
#1817=ELLIPSE('',#106766,0.354421121839405,0.321488565205236);
#1818=ELLIPSE('',#106768,0.472048618674185,0.428376333588625);
#1819=ELLIPSE('',#106769,0.472049204212207,0.428376856670675);
#1820=ELLIPSE('',#106770,0.354421145890722,0.321488604122502);
#1821=ELLIPSE('',#106771,0.354421089420675,0.321488612084178);
#1822=ELLIPSE('',#106776,0.472049204512402,0.428376857315463);
#1823=ELLIPSE('',#106777,0.47204861839104,0.428376332980329);
#1824=ELLIPSE('',#106778,0.354420976863445,0.321488380354816);
#1825=ELLIPSE('',#106779,0.354421121834752,0.321488565196016);
#1826=ELLIPSE('',#106781,0.472048618673901,0.428376333588);
#1827=ELLIPSE('',#106782,0.472049204214096,0.428376856674452);
#1828=ELLIPSE('',#106783,0.354421145894766,0.321488604130566);
#1829=ELLIPSE('',#106784,0.354421089421831,0.321488612086608);
#1830=ELLIPSE('',#106789,0.472049204510581,0.428376857311865);
#1831=ELLIPSE('',#106790,0.472048618391265,0.42837633298078);
#1832=ELLIPSE('',#106791,0.354420976864482,0.321488380356888);
#1833=ELLIPSE('',#106792,0.354421121837425,0.32148856520138);
#1834=ELLIPSE('',#106794,0.472048618673329,0.42837633358685);
#1835=ELLIPSE('',#106795,0.472049204213157,0.428376856672562);
#1836=ELLIPSE('',#106796,0.354421145894411,0.321488604129916);
#1837=ELLIPSE('',#106797,0.354421089422569,0.321488612087967);
#1838=ELLIPSE('',#106802,0.472049204510999,0.428376857312677);
#1839=ELLIPSE('',#106803,0.472048618392686,0.428376332983611);
#1840=ELLIPSE('',#106804,0.354420976865054,0.32148838035797);
#1841=ELLIPSE('',#106805,0.354421121835212,0.321488565196872);
#1842=ELLIPSE('',#106807,0.472048618672229,0.428376333584709);
#1843=ELLIPSE('',#106808,0.47204920421317,0.428376856672604);
#1844=ELLIPSE('',#106809,0.354421145893081,0.321488604127171);
#1845=ELLIPSE('',#106810,0.354421089422993,0.321488612088897);
#1846=ELLIPSE('',#106815,0.472049204511446,0.428376857313571);
#1847=ELLIPSE('',#106816,0.472048618393155,0.428376332984517);
#1848=ELLIPSE('',#106817,0.354420976864664,0.321488380357234);
#1849=ELLIPSE('',#106818,0.354421121834986,0.321488565196496);
#1850=ELLIPSE('',#106820,0.472048618673363,0.428376333586959);
#1851=ELLIPSE('',#106821,0.472049204211319,0.428376856668897);
#1852=ELLIPSE('',#106822,0.354421145892422,0.32148860412587);
#1853=ELLIPSE('',#106823,0.354421089420983,0.321488612084892);
#1854=ELLIPSE('',#106828,0.472049204511805,0.428376857314261);
#1855=ELLIPSE('',#106829,0.472048618392444,0.428376332983087);
#1856=ELLIPSE('',#106830,0.354420976864753,0.321488380357426);
#1857=ELLIPSE('',#106831,0.354421121834726,0.321488565195851);
#1858=ELLIPSE('',#106833,0.472048618672876,0.428376333585999);
#1859=ELLIPSE('',#106834,0.472049204213336,0.428376856672891);
#1860=ELLIPSE('',#106835,0.354421145892402,0.321488604125789);
#1861=ELLIPSE('',#106836,0.354421089422495,0.321488612087972);
#1862=ELLIPSE('',#106841,0.47204920451177,0.428376857314165);
#1863=ELLIPSE('',#106842,0.472048618392473,0.42837633298315);
#1864=ELLIPSE('',#106843,0.354420976864884,0.321488380357631);
#1865=ELLIPSE('',#106844,0.354421121836591,0.321488565199702);
#1866=ELLIPSE('',#106846,0.472048618674066,0.428376333588222);
#1867=ELLIPSE('',#106847,0.472049204213538,0.428376856673325);
#1868=ELLIPSE('',#106848,0.354421145892755,0.321488604126568);
#1869=ELLIPSE('',#106849,0.354421089419435,0.321488612081731);
#1870=ELLIPSE('',#106854,0.472049204511611,0.428376857313908);
#1871=ELLIPSE('',#106855,0.472048618391763,0.428376332981745);
#1872=ELLIPSE('',#106856,0.354420976865304,0.321488380358487);
#1873=ELLIPSE('',#106857,0.354421121837747,0.321488565201944);
#1874=ELLIPSE('',#106859,0.472048618672451,0.428376333585147);
#1875=ELLIPSE('',#106860,0.47204920421305,0.428376856672371);
#1876=ELLIPSE('',#106861,0.354421145893108,0.321488604127281);
#1877=ELLIPSE('',#106862,0.354421089420954,0.32148861208485);
#1878=ELLIPSE('',#106867,0.472049204509719,0.428376857310066);
#1879=ELLIPSE('',#106868,0.472048618392744,0.428376332983729);
#1880=ELLIPSE('',#106869,0.354420976866554,0.321488380361071);
#1881=ELLIPSE('',#106870,0.354421121835452,0.321488565197322);
#1882=ELLIPSE('',#106872,0.472048618672175,0.428376333584535);
#1883=ELLIPSE('',#106873,0.472049204213562,0.428376856673388);
#1884=ELLIPSE('',#106874,0.354421145891911,0.321488604124825);
#1885=ELLIPSE('',#106875,0.354421089423445,0.321488612089755);
#1886=ELLIPSE('',#106880,0.472049204511528,0.428376857313709);
#1887=ELLIPSE('',#106881,0.472048618393424,0.42837633298505);
#1888=ELLIPSE('',#106882,0.354420976866572,0.321488380361074);
#1889=ELLIPSE('',#106883,0.354421121834629,0.321488565195727);
#1890=ELLIPSE('',#106885,0.472048618671858,0.428376333583949);
#1891=ELLIPSE('',#106886,0.472049204212922,0.42837685667212);
#1892=ELLIPSE('',#106887,0.354421145894853,0.321488604130806);
#1893=ELLIPSE('',#106888,0.354421089421859,0.321488612086603);
#1894=ELLIPSE('',#106893,0.472049204510708,0.428376857312109);
#1895=ELLIPSE('',#106894,0.472048618392905,0.428376332983962);
#1896=ELLIPSE('',#106895,0.354420976864336,0.321488380356588);
#1897=ELLIPSE('',#106896,0.354421121837681,0.321488565201792);
#1898=ELLIPSE('',#106898,0.47204861867398,0.428376333588129);
#1899=ELLIPSE('',#106899,0.472049204212391,0.42837685667103);
#1900=ELLIPSE('',#106900,0.354421145891274,0.321488604123569);
#1901=ELLIPSE('',#106901,0.354421089422014,0.321488612086951);
#1902=ELLIPSE('',#106906,0.472049204509829,0.428376857310356);
#1903=ELLIPSE('',#106907,0.47204861839254,0.428376332983332);
#1904=ELLIPSE('',#106908,0.354420976864865,0.321488380357682);
#1905=ELLIPSE('',#106909,0.354421121834297,0.321488565195027);
#1906=ELLIPSE('',#106911,0.472048618674307,0.428376333588772);
#1907=ELLIPSE('',#106912,0.472049204212345,0.42837685667097);
#1908=ELLIPSE('',#106913,0.354421145891073,0.321488604123106);
#1909=ELLIPSE('',#106914,0.354421089421874,0.321488612086676);
#1910=ELLIPSE('',#106919,0.472049204509867,0.428376857310419);
#1911=ELLIPSE('',#106920,0.472048618391784,0.428376332981756);
#1912=ELLIPSE('',#106921,0.354420976863024,0.321488380353946);
#1913=ELLIPSE('',#106922,0.354421121836327,0.321488565199162);
#1914=ELLIPSE('',#106924,0.472048618674761,0.428376333589649);
#1915=ELLIPSE('',#106925,0.472049204213332,0.428376856672879);
#1916=ELLIPSE('',#106926,0.354421145895874,0.321488604132804);
#1917=ELLIPSE('',#106927,0.354421089422406,0.321488612087776);
#1918=ELLIPSE('',#106932,0.472049204510431,0.428376857311526);
#1919=ELLIPSE('',#106933,0.472048618392641,0.428376332983465);
#1920=ELLIPSE('',#106934,0.354420976866106,0.321488380360133);
#1921=ELLIPSE('',#106935,0.354421121836792,0.321488565199963);
#1922=ELLIPSE('',#106937,0.472048618673813,0.428376333587806);
#1923=ELLIPSE('',#106938,0.472049204213194,0.428376856672618);
#1924=ELLIPSE('',#106939,0.354421145892162,0.321488604125355);
#1925=ELLIPSE('',#106940,0.35442108942166,0.321488612086207);
#1926=ELLIPSE('',#106945,0.472049204510832,0.428376857312327);
#1927=ELLIPSE('',#106946,0.472048618391221,0.428376332980707);
#1928=ELLIPSE('',#106947,0.35442097686472,0.321488380357379);
#1929=ELLIPSE('',#106948,0.35442112183282,0.321488565192222);
#1930=ELLIPSE('',#106950,0.472048618672444,0.428376333585101);
#1931=ELLIPSE('',#106951,0.472049204212583,0.428376856671445);
#1932=ELLIPSE('',#106952,0.354421145893025,0.321488604127087);
#1933=ELLIPSE('',#106953,0.35442108942345,0.321488612089842);
#1934=ELLIPSE('',#106958,0.472049204511797,0.428376857314251);
#1935=ELLIPSE('',#106959,0.472048618392414,0.428376332983038);
#1936=ELLIPSE('',#106960,0.354420976864875,0.321488380357668);
#1937=ELLIPSE('',#106961,0.354421121834933,0.321488565196381);
#1938=ELLIPSE('',#106963,0.472048618671548,0.428376333583326);
#1939=ELLIPSE('',#106964,0.472049204213259,0.428376856672769);
#1940=ELLIPSE('',#106965,0.354421145891538,0.321488604124113);
#1941=ELLIPSE('',#106966,0.354421089423352,0.321488612089676);
#1942=ELLIPSE('',#106971,0.47204920451107,0.428376857312751);
#1943=ELLIPSE('',#106972,0.472048618390752,0.428376332979759);
#1944=ELLIPSE('',#106973,0.354420976865788,0.321488380359456);
#1945=ELLIPSE('',#106974,0.354421121838495,0.321488565203415);
#1946=ELLIPSE('',#106976,0.472048618672205,0.42837633358462);
#1947=ELLIPSE('',#106977,0.472049204213218,0.428376856672709);
#1948=ELLIPSE('',#106978,0.354421145888541,0.321488604118161);
#1949=ELLIPSE('',#106979,0.354421089422543,0.321488612087925);
#1950=ELLIPSE('',#106984,0.472049204511644,0.428376857313924);
#1951=ELLIPSE('',#106985,0.472048618391977,0.428376332982213);
#1952=ELLIPSE('',#106986,0.354420976865027,0.32148838035787);
#1953=ELLIPSE('',#106987,0.35442112183701,0.321488565200554);
#1954=ELLIPSE('',#106989,0.472048618674897,0.428376333589962);
#1955=ELLIPSE('',#106990,0.472049204212709,0.428376856671672);
#1956=ELLIPSE('',#106991,0.354421145893339,0.321488604127641);
#1957=ELLIPSE('',#106992,0.354421089420524,0.321488612084021);
#1958=ELLIPSE('',#106997,0.472049204511113,0.428376857312905);
#1959=ELLIPSE('',#106998,0.472048618391887,0.42837633298201);
#1960=ELLIPSE('',#106999,0.354420976864428,0.32148838035676);
#1961=ELLIPSE('',#107000,0.354421121836451,0.321488565199322);
#1962=ELLIPSE('',#107002,0.472048618673337,0.428376333586849);
#1963=ELLIPSE('',#107003,0.472049204213993,0.42837685667426);
#1964=ELLIPSE('',#107004,0.354421145891899,0.321488604124793);
#1965=ELLIPSE('',#107005,0.354421089420731,0.32148861208434);
#1966=ELLIPSE('',#107010,0.472049204511345,0.428376857313415);
#1967=ELLIPSE('',#107011,0.472048618393512,0.428376332985235);
#1968=ELLIPSE('',#107012,0.354420976865338,0.321488380358552);
#1969=ELLIPSE('',#107013,0.354421121834909,0.321488565196267);
#1970=ELLIPSE('',#107015,0.472048618673628,0.428376333587382);
#1971=ELLIPSE('',#107016,0.472049204212025,0.428376856670342);
#1972=ELLIPSE('',#107017,0.354421145891821,0.321488604124643);
#1973=ELLIPSE('',#107018,0.354421089423547,0.32148861209004);
#1974=ELLIPSE('',#107023,0.472049204511327,0.428376857313316);
#1975=ELLIPSE('',#107024,0.472048618392492,0.428376332983142);
#1976=ELLIPSE('',#107025,0.354420976864652,0.321488380357205);
#1977=ELLIPSE('',#107026,0.354421121836402,0.321488565199307);
#1978=ELLIPSE('',#107028,0.472048618674604,0.42837633358946);
#1979=ELLIPSE('',#107029,0.472049204212897,0.428376856672065);
#1980=ELLIPSE('',#107030,0.354421145891663,0.321488604124326);
#1981=ELLIPSE('',#107031,0.354421089422031,0.321488612086993);
#1982=ELLIPSE('',#107036,0.472049204509891,0.428376857310496);
#1983=ELLIPSE('',#107037,0.472048618391715,0.428376332981714);
#1984=ELLIPSE('',#107038,0.354420976865568,0.321488380359037);
#1985=ELLIPSE('',#107039,0.35442112183639,0.321488565199294);
#1986=ELLIPSE('',#107041,0.472048618673416,0.428376333587058);
#1987=ELLIPSE('',#107042,0.472049204212742,0.428376856671765);
#1988=ELLIPSE('',#107043,0.354421145896618,0.321488604134214);
#1989=ELLIPSE('',#107044,0.354421089421241,0.321488612085355);
#1990=ELLIPSE('',#107049,0.472049204511421,0.428376857313551);
#1991=ELLIPSE('',#107050,0.472048618392505,0.428376332983233);
#1992=ELLIPSE('',#107051,0.354420976863069,0.321488380353995);
#1993=ELLIPSE('',#107052,0.35442112183516,0.321488565196781);
#1994=ELLIPSE('',#107054,0.472048618673188,0.428376333586607);
#1995=ELLIPSE('',#107055,0.472049204213191,0.428376856672666);
#1996=ELLIPSE('',#107056,0.354421145891334,0.321488604123686);
#1997=ELLIPSE('',#107057,0.354421089420386,0.321488612083722);
#1998=ELLIPSE('',#107062,0.472049204510831,0.428376857312323);
#1999=ELLIPSE('',#107063,0.472048618392,0.428376332982215);
#2000=ELLIPSE('',#107064,0.354420976865575,0.32148838035904);
#2001=ELLIPSE('',#107065,0.354421121833158,0.321488565192756);
#2002=ELLIPSE('',#107067,0.472048618673296,0.428376333586792);
#2003=ELLIPSE('',#107068,0.472049204211677,0.428376856669657);
#2004=ELLIPSE('',#107069,0.354421145893456,0.321488604128007);
#2005=ELLIPSE('',#107070,0.354421089420597,0.321488612084059);
#2006=ELLIPSE('',#107075,0.472049204510519,0.428376857311711);
#2007=ELLIPSE('',#107076,0.472048618393586,0.428376332985414);
#2008=ELLIPSE('',#107077,0.354420976863066,0.321488380354067);
#2009=ELLIPSE('',#107078,0.3544211218372,0.321488565200811);
#2010=ELLIPSE('',#107080,0.472048618673438,0.428376333587092);
#2011=ELLIPSE('',#107081,0.472049204211534,0.428376856669341);
#2012=ELLIPSE('',#107082,0.354421145896177,0.321488604133354);
#2013=ELLIPSE('',#107083,0.354421089423546,0.321488612089943);
#2014=ELLIPSE('',#107088,0.472049204511482,0.428376857313627);
#2015=ELLIPSE('',#107089,0.472048618392421,0.428376332983089);
#2016=ELLIPSE('',#107090,0.354420976866456,0.321488380360847);
#2017=ELLIPSE('',#107091,0.354421121834971,0.32148856519634);
#2018=ELLIPSE('',#107093,0.47204861867389,0.428376333587944);
#2019=ELLIPSE('',#107094,0.472049204213437,0.4283768566731);
#2020=ELLIPSE('',#107095,0.35442114589374,0.321488604128488);
#2021=ELLIPSE('',#107096,0.354421089423662,0.321488612090211);
#2022=ELLIPSE('',#107099,0.472049204511149,0.428376857312952);
#2023=ELLIPSE('',#107100,0.472048618391616,0.428376332981492);
#2024=ELLIPSE('',#107101,0.354420976863965,0.321488380355734);
#2025=ELLIPSE('',#107102,0.354421121839368,0.3214885652052);
#2026=ELLIPSE('',#107104,0.472048618673971,0.428376333588171);
#2027=ELLIPSE('',#107105,0.472049204213616,0.428376856673503);
#2028=ELLIPSE('',#107106,0.354421145894116,0.321488604129308);
#2029=ELLIPSE('',#107107,0.354421089421021,0.321488612084896);
#2030=ELLIPSE('',#107112,0.472049204511451,0.428376857313542);
#2031=ELLIPSE('',#107113,0.472048618392002,0.428376332982204);
#2032=ELLIPSE('',#107114,0.354420976865778,0.32148838035945);
#2033=ELLIPSE('',#107115,0.354421121835973,0.321488565198471);
#2034=ELLIPSE('',#107117,0.472048618674194,0.428376333588553);
#2035=ELLIPSE('',#107118,0.472049204212065,0.428376856670387);
#2036=ELLIPSE('',#107119,0.354421145894391,0.321488604129854);
#2037=ELLIPSE('',#107120,0.354421089422029,0.321488612087025);
#2038=ELLIPSE('',#107125,0.472049204511657,0.428376857313933);
#2039=ELLIPSE('',#107126,0.472048618391513,0.428376332981293);
#2040=ELLIPSE('',#107127,0.354420976864311,0.321488380356496);
#2041=ELLIPSE('',#107128,0.354421121837407,0.321488565201336);
#2042=ELLIPSE('',#107130,0.472048618672929,0.42837633358606);
#2043=ELLIPSE('',#107131,0.472049204212117,0.428376856670511);
#2044=ELLIPSE('',#107132,0.354421145894905,0.321488604130814);
#2045=ELLIPSE('',#107133,0.354421089422112,0.321488612087143);
#2046=ELLIPSE('',#107138,0.472049204511992,0.428376857314651);
#2047=ELLIPSE('',#107139,0.472048618392913,0.428376332984082);
#2048=ELLIPSE('',#107140,0.354420976865269,0.321488380358449);
#2049=ELLIPSE('',#107141,0.354421121834688,0.321488565195839);
#2050=ELLIPSE('',#107143,0.472048618673509,0.428376333587237);
#2051=ELLIPSE('',#107144,0.472049204213274,0.428376856672824);
#2052=ELLIPSE('',#107145,0.354421145892845,0.321488604126746);
#2053=ELLIPSE('',#107146,0.354421089425724,0.321488612094367);
#2054=ELLIPSE('',#107151,0.472049204511633,0.428376857313873);
#2055=ELLIPSE('',#107152,0.472048618392605,0.428376332983422);
#2056=ELLIPSE('',#107153,0.354420976864453,0.321488380356726);
#2057=ELLIPSE('',#107154,0.354421121832141,0.321488565190751);
#2058=ELLIPSE('',#107156,0.472048618673539,0.428376333587287);
#2059=ELLIPSE('',#107157,0.472049204213293,0.428376856672817);
#2060=ELLIPSE('',#107158,0.354421145894062,0.321488604129175);
#2061=ELLIPSE('',#107159,0.354421089419115,0.321488612081158);
#2062=ELLIPSE('',#107164,0.472049204511243,0.428376857313128);
#2063=ELLIPSE('',#107165,0.472048618391538,0.428376332981319);
#2064=ELLIPSE('',#107166,0.354420976864454,0.3214883803568);
#2065=ELLIPSE('',#107167,0.354421121833766,0.321488565193981);
#2066=ELLIPSE('',#107169,0.47204861867417,0.428376333588541);
#2067=ELLIPSE('',#107170,0.472049204213016,0.428376856672282);
#2068=ELLIPSE('',#107171,0.354421145891356,0.321488604123696);
#2069=ELLIPSE('',#107172,0.354421089423352,0.321488612089603);
#2070=ELLIPSE('',#107177,0.47204920451092,0.428376857312493);
#2071=ELLIPSE('',#107178,0.472048618392258,0.428376332982749);
#2072=ELLIPSE('',#107179,0.354420976865082,0.321488380358088);
#2073=ELLIPSE('',#107180,0.354421121835669,0.321488565197869);
#2074=ELLIPSE('',#107182,0.472048618673151,0.428376333586468);
#2075=ELLIPSE('',#107183,0.472049204211844,0.428376856669944);
#2076=ELLIPSE('',#107184,0.354421145894343,0.321488604129742);
#2077=ELLIPSE('',#107185,0.354421089422269,0.321488612087402);
#2078=ELLIPSE('',#107190,0.472049204508892,0.428376857308545);
#2079=ELLIPSE('',#107191,0.472048618392121,0.42837633298247);
#2080=ELLIPSE('',#107192,0.354420976863941,0.321488380355759);
#2081=ELLIPSE('',#107193,0.354421121837472,0.32148856520146);
#2082=ELLIPSE('',#107195,0.472048618672543,0.428376333585301);
#2083=ELLIPSE('',#107196,0.472049204213821,0.428376856673893);
#2084=ELLIPSE('',#107197,0.35442114589205,0.321488604125153);
#2085=ELLIPSE('',#107198,0.354421089420019,0.321488612082947);
#2086=ELLIPSE('',#107203,0.472049204511413,0.42837685731347);
#2087=ELLIPSE('',#107204,0.472048618392691,0.428376332983646);
#2088=ELLIPSE('',#107205,0.354420976864115,0.321488380356169);
#2089=ELLIPSE('',#107206,0.354421121832944,0.321488565192392);
#2090=ELLIPSE('',#107208,0.472048618674026,0.428376333588235);
#2091=ELLIPSE('',#107209,0.472049204212005,0.428376856670295);
#2092=ELLIPSE('',#107210,0.354421145892444,0.321488604125956);
#2093=ELLIPSE('',#107211,0.35442108942116,0.321488612085219);
#2094=ELLIPSE('',#107216,0.47204920450981,0.428376857310287);
#2095=ELLIPSE('',#107217,0.472048618392289,0.428376332982821);
#2096=ELLIPSE('',#107218,0.354420976862782,0.321488380353437);
#2097=ELLIPSE('',#107219,0.354421121836506,0.321488565199431);
#2098=ELLIPSE('',#107221,0.472048618672653,0.42837633358548);
#2099=ELLIPSE('',#107222,0.472049204213736,0.428376856673694);
#2100=ELLIPSE('',#107223,0.354421145890053,0.321488604121152);
#2101=ELLIPSE('',#107224,0.354421089423222,0.321488612089361);
#2102=ELLIPSE('',#107229,0.472049204509417,0.428376857309544);
#2103=ELLIPSE('',#107230,0.472048618391604,0.428376332981422);
#2104=ELLIPSE('',#107231,0.354420976862723,0.321488380353292);
#2105=ELLIPSE('',#107232,0.354421121837083,0.32148856520067);
#2106=ELLIPSE('',#107234,0.47204861867469,0.428376333589523);
#2107=ELLIPSE('',#107235,0.47204920421263,0.428376856671494);
#2108=ELLIPSE('',#107236,0.354421145893487,0.321488604127993);
#2109=ELLIPSE('',#107237,0.354421089421634,0.321488612086208);
#2110=ELLIPSE('',#107242,0.47204920450963,0.428376857309992);
#2111=ELLIPSE('',#107243,0.472048618392772,0.428376332983745);
#2112=ELLIPSE('',#107244,0.354420976863782,0.321488380355444);
#2113=ELLIPSE('',#107245,0.354421121836615,0.321488565199704);
#2114=ELLIPSE('',#107247,0.47204861867308,0.428376333586376);
#2115=ELLIPSE('',#107248,0.472049204212482,0.428376856671214);
#2116=ELLIPSE('',#107249,0.354421145892683,0.321488604126402);
#2117=ELLIPSE('',#107250,0.35442108942268,0.321488612088291);
#2118=ELLIPSE('',#107255,0.472049204510717,0.428376857312061);
#2119=ELLIPSE('',#107256,0.472048618391451,0.428376332981167);
#2120=ELLIPSE('',#107257,0.354420976866113,0.321488380360137);
#2121=ELLIPSE('',#107258,0.354421121835235,0.321488565196901);
#2122=ELLIPSE('',#107260,0.4720486186743,0.428376333588738);
#2123=ELLIPSE('',#107261,0.472049204212938,0.428376856672103);
#2124=ELLIPSE('',#107262,0.354421145893203,0.321488604127511);
#2125=ELLIPSE('',#107263,0.354421089424015,0.321488612090953);
#2126=ELLIPSE('',#107268,0.472049204511672,0.428376857313994);
#2127=ELLIPSE('',#107269,0.472048618392936,0.428376332984117);
#2128=ELLIPSE('',#107270,0.354420976863078,0.321488380353981);
#2129=ELLIPSE('',#107271,0.354421121835837,0.321488565198135);
#2130=ELLIPSE('',#107273,0.4720486186744,0.428376333588985);
#2131=ELLIPSE('',#107274,0.472049204212671,0.428376856671578);
#2132=ELLIPSE('',#107275,0.354421145894098,0.321488604129234);
#2133=ELLIPSE('',#107276,0.354421089421883,0.321488612086657);
#2134=ELLIPSE('',#107281,0.472049204510614,0.428376857311898);
#2135=ELLIPSE('',#107282,0.472048618393337,0.428376332984887);
#2136=ELLIPSE('',#107283,0.354420976865991,0.321488380359936);
#2137=ELLIPSE('',#107284,0.354421121835589,0.321488565197568);
#2138=ELLIPSE('',#107286,0.472048618674229,0.428376333588641);
#2139=ELLIPSE('',#107287,0.472049204213025,0.42837685667231);
#2140=ELLIPSE('',#107288,0.35442114589626,0.321488604133465);
#2141=ELLIPSE('',#107289,0.35442108942249,0.321488612087879);
#2142=ELLIPSE('',#107292,0.472049204511229,0.428376857313123);
#2143=ELLIPSE('',#107293,0.47204861839257,0.428376332983376);
#2144=ELLIPSE('',#107294,0.354420976864408,0.321488380356651);
#2145=ELLIPSE('',#107295,0.354421121838439,0.321488565203349);
#2146=ELLIPSE('',#107297,0.472048618674394,0.428376333588988);
#2147=ELLIPSE('',#107298,0.472049204213168,0.428376856672599);
#2148=ELLIPSE('',#107299,0.354421145893815,0.321488604128643);
#2149=ELLIPSE('',#107300,0.354421089424289,0.321488612091436);
#2150=ELLIPSE('',#107305,0.472049204513252,0.42837685731712);
#2151=ELLIPSE('',#107306,0.472048618392165,0.428376332982546);
#2152=ELLIPSE('',#107307,0.35442097686289,0.321488380353694);
#2153=ELLIPSE('',#107308,0.354421121835997,0.321488565198458);
#2154=ELLIPSE('',#107310,0.472048618674151,0.428376333588511);
#2155=ELLIPSE('',#107311,0.472049204211785,0.428376856669885);
#2156=ELLIPSE('',#107312,0.354421145894632,0.321488604130297);
#2157=ELLIPSE('',#107313,0.354421089422824,0.321488612088477);
#2158=ELLIPSE('',#107318,0.472049204511394,0.428376857313407);
#2159=ELLIPSE('',#107319,0.472048618391184,0.428376332980646);
#2160=ELLIPSE('',#107320,0.354420976864394,0.32148838035678);
#2161=ELLIPSE('',#107321,0.354421121834998,0.321488565196511);
#2162=ELLIPSE('',#107323,0.472048618674661,0.428376333589502);
#2163=ELLIPSE('',#107324,0.472049204212487,0.428376856671257);
#2164=ELLIPSE('',#107325,0.354421145891117,0.321488604123307);
#2165=ELLIPSE('',#107326,0.354421089423795,0.321488612090472);
#2166=ELLIPSE('',#107331,0.472049204510894,0.428376857312474);
#2167=ELLIPSE('',#107332,0.472048618391186,0.428376332980609);
#2168=ELLIPSE('',#107333,0.354420976865725,0.321488380359322);
#2169=ELLIPSE('',#107334,0.354421121834588,0.321488565195654);
#2170=ELLIPSE('',#107336,0.472048618673108,0.428376333586399);
#2171=ELLIPSE('',#107337,0.472049204212361,0.428376856671049);
#2172=ELLIPSE('',#107338,0.354421145893163,0.321488604127362);
#2173=ELLIPSE('',#107339,0.354421089423452,0.321488612089836);
#2174=ELLIPSE('',#107344,0.472049204511179,0.428376857313092);
#2175=ELLIPSE('',#107345,0.472048618392961,0.42837633298412);
#2176=ELLIPSE('',#107346,0.354420976863802,0.321488380355433);
#2177=ELLIPSE('',#107347,0.354421121837851,0.321488565202186);
#2178=ELLIPSE('',#107349,0.472048618671871,0.428376333583965);
#2179=ELLIPSE('',#107350,0.472049204211579,0.428376856669446);
#2180=ELLIPSE('',#107351,0.35442114589121,0.32148860412345);
#2181=ELLIPSE('',#107352,0.354421089421435,0.321488612085847);
#2182=ELLIPSE('',#107357,0.472049204511322,0.428376857313307);
#2183=ELLIPSE('',#107358,0.472048618391922,0.428376332982069);
#2184=ELLIPSE('',#107359,0.354420976865897,0.321488380359689);
#2185=ELLIPSE('',#107360,0.35442112183738,0.321488565201278);
#2186=ELLIPSE('',#107362,0.472048618674387,0.428376333588996);
#2187=ELLIPSE('',#107363,0.472049204212476,0.428376856671206);
#2188=ELLIPSE('',#107364,0.354421145894326,0.321488604129683);
#2189=ELLIPSE('',#107365,0.3544210894222,0.321488612087341);
#2190=ELLIPSE('',#107370,0.472049204510946,0.428376857312566);
#2191=ELLIPSE('',#107371,0.472048618391712,0.428376332981558);
#2192=ELLIPSE('',#107372,0.354420976866645,0.321488380361217);
#2193=ELLIPSE('',#107373,0.354421121838504,0.321488565203492);
#2194=ELLIPSE('',#107375,0.472048618673501,0.428376333587255);
#2195=ELLIPSE('',#107376,0.472049204212708,0.428376856671664);
#2196=ELLIPSE('',#107377,0.35442114589414,0.321488604129325);
#2197=ELLIPSE('',#107378,0.354421089422287,0.321488612087437);
#2198=ELLIPSE('',#107383,0.472049204511479,0.42837685731363);
#2199=ELLIPSE('',#107384,0.472048618391853,0.428376332981929);
#2200=ELLIPSE('',#107385,0.354420976866264,0.321488380360526);
#2201=ELLIPSE('',#107386,0.354421121836331,0.321488565199092);
#2202=ELLIPSE('',#107388,0.472048618675346,0.428376333590846);
#2203=ELLIPSE('',#107389,0.47204920421198,0.428376856670232);
#2204=ELLIPSE('',#107390,0.354421145889929,0.321488604120882);
#2205=ELLIPSE('',#107391,0.354421089421345,0.321488612085622);
#2206=ELLIPSE('',#107396,0.472049204509595,0.428376857309901);
#2207=ELLIPSE('',#107397,0.472048618392921,0.428376332984105);
#2208=ELLIPSE('',#107398,0.35442097686446,0.321488380356807);
#2209=ELLIPSE('',#107399,0.35442112183345,0.32148856519335);
#2210=ELLIPSE('',#107401,0.472048618672761,0.428376333585721);
#2211=ELLIPSE('',#107402,0.472049204211995,0.428376856670272);
#2212=ELLIPSE('',#107403,0.354421145890888,0.321488604122831);
#2213=ELLIPSE('',#107404,0.354421089421532,0.321488612085962);
#2214=ELLIPSE('',#107409,0.472049204511288,0.428376857313216);
#2215=ELLIPSE('',#107410,0.472048618391648,0.428376332981492);
#2216=ELLIPSE('',#107411,0.354420976864546,0.321488380357008);
#2217=ELLIPSE('',#107412,0.354421121836294,0.321488565198935);
#2218=ELLIPSE('',#107414,0.472048618674408,0.428376333588983);
#2219=ELLIPSE('',#107415,0.472049204211926,0.428376856670145);
#2220=ELLIPSE('',#107416,0.354421145893214,0.321488604127459);
#2221=ELLIPSE('',#107417,0.354421089423539,0.321488612089965);
#2222=ELLIPSE('',#107422,0.472049204510058,0.428376857310839);
#2223=ELLIPSE('',#107423,0.472048618393402,0.428376332984991);
#2224=ELLIPSE('',#107424,0.354420976865732,0.321488380359386);
#2225=ELLIPSE('',#107425,0.354421121836976,0.321488565200376);
#2226=ELLIPSE('',#107427,0.472048618673465,0.428376333587143);
#2227=ELLIPSE('',#107428,0.472049204213126,0.428376856672526);
#2228=ELLIPSE('',#107429,0.354421145890888,0.321488604122835);
#2229=ELLIPSE('',#107430,0.354421089422305,0.321488612087484);
#2230=ELLIPSE('',#107435,0.472049204511117,0.428376857312922);
#2231=ELLIPSE('',#107436,0.47204861839179,0.428376332981839);
#2232=ELLIPSE('',#107437,0.35442097686677,0.321488380361499);
#2233=ELLIPSE('',#107438,0.354421121836319,0.321488565199035);
#2234=ELLIPSE('',#107440,0.472048618674479,0.428376333589128);
#2235=ELLIPSE('',#107441,0.47204920421329,0.428376856672826);
#2236=ELLIPSE('',#107442,0.354421145894268,0.321488604129596);
#2237=ELLIPSE('',#107443,0.354421089422428,0.321488612087792);
#2238=ELLIPSE('',#107448,0.472049204510683,0.428376857312038);
#2239=ELLIPSE('',#107449,0.472048618393508,0.428376332985237);
#2240=ELLIPSE('',#107450,0.354420976865022,0.32148838035803);
#2241=ELLIPSE('',#107451,0.354421121835537,0.321488565197519);
#2242=ELLIPSE('',#107453,0.472048618673479,0.428376333587187);
#2243=ELLIPSE('',#107454,0.472049204211936,0.428376856670164);
#2244=ELLIPSE('',#107455,0.354421145892554,0.321488604126193);
#2245=ELLIPSE('',#107456,0.354421089420411,0.3214886120837);
#2246=ELLIPSE('',#107461,0.472049204511685,0.428376857314037);
#2247=ELLIPSE('',#107462,0.47204861839225,0.428376332982777);
#2248=ELLIPSE('',#107463,0.354420976864416,0.321488380356758);
#2249=ELLIPSE('',#107464,0.354421121837932,0.321488565202383);
#2250=ELLIPSE('',#107466,0.472048618673388,0.428376333586979);
#2251=ELLIPSE('',#107467,0.472049204211487,0.42837685666926);
#2252=ELLIPSE('',#107468,0.354421145894157,0.32148860412932);
#2253=ELLIPSE('',#107469,0.354421089422988,0.321488612088863);
#2254=ELLIPSE('',#107474,0.472049204510669,0.428376857312049);
#2255=ELLIPSE('',#107475,0.472048618393432,0.428376332985066);
#2256=ELLIPSE('',#107476,0.354420976864168,0.321488380356288);
#2257=ELLIPSE('',#107477,0.354421121837713,0.321488565201861);
#2258=ELLIPSE('',#107479,0.472048618673566,0.428376333587318);
#2259=ELLIPSE('',#107480,0.472049204212713,0.428376856671703);
#2260=ELLIPSE('',#107481,0.354421145892746,0.32148860412653);
#2261=ELLIPSE('',#107482,0.354421089422267,0.321488612087543);
#2262=ELLIPSE('',#107602,0.146692861885778,0.127051669378566);
#2263=ELLIPSE('',#107614,0.146691465566803,0.127050784763753);
#2264=ELLIPSE('',#107631,0.146692861886413,0.127051669378057);
#2265=ELLIPSE('',#107642,0.14669146556691,0.12705078476387);
#2266=ELLIPSE('',#107646,0.146692861887922,0.127051669380119);
#2267=ELLIPSE('',#107658,0.14669146556702,0.127050784764041);
#2268=ELLIPSE('',#107675,0.146692861887039,0.127051669380184);
#2269=ELLIPSE('',#107686,0.146691465566734,0.12705078476371);
#2270=ELLIPSE('',#107690,0.146692861889571,0.127051669380672);
#2271=ELLIPSE('',#107702,0.146691465567211,0.127050784764187);
#2272=ELLIPSE('',#107719,0.146692861887923,0.127051669379853);
#2273=ELLIPSE('',#107730,0.146691465566873,0.127050784763828);
#2274=ELLIPSE('',#107734,0.146692861885695,0.127051669378166);
#2275=ELLIPSE('',#107746,0.146691465566617,0.127050784763644);
#2276=ELLIPSE('',#107763,0.146692861890006,0.12705166938115);
#2277=ELLIPSE('',#107774,0.146691465566989,0.127050784763962);
#2278=ELLIPSE('',#107778,0.146692861886538,0.127051669378574);
#2279=ELLIPSE('',#107790,0.146691465566865,0.127050784763831);
#2280=ELLIPSE('',#107807,0.146692861888534,0.127051669379887);
#2281=ELLIPSE('',#107818,0.14669146556704,0.127050784763975);
#2282=ELLIPSE('',#107822,0.14669286189017,0.127051669381253);
#2283=ELLIPSE('',#107834,0.146691465566333,0.127050784763404);
#2284=ELLIPSE('',#107851,0.146692861888775,0.127051669381276);
#2285=ELLIPSE('',#107862,0.146691465566996,0.127050784763966);
#2286=ELLIPSE('',#107866,0.146692861889956,0.127051669380713);
#2287=ELLIPSE('',#107878,0.146691465567727,0.127050784764622);
#2288=ELLIPSE('',#107895,0.146692861890152,0.127051669381072);
#2289=ELLIPSE('',#107906,0.146691465566229,0.127050784763335);
#2290=ELLIPSE('',#107910,0.146692861889335,0.127051669380942);
#2291=ELLIPSE('',#107922,0.146691465567614,0.127050784764493);
#2292=ELLIPSE('',#107939,0.146692861888875,0.127051669380474);
#2293=ELLIPSE('',#107950,0.146691465567108,0.127050784764015);
#2294=ELLIPSE('',#107954,0.146692861889473,0.127051669380558);
#2295=ELLIPSE('',#107966,0.146691465566935,0.127050784763893);
#2296=ELLIPSE('',#107983,0.146692861888244,0.127051669380723);
#2297=ELLIPSE('',#107994,0.14669146556749,0.127050784764377);
#2298=ELLIPSE('',#107998,0.14669286188738,0.12705166938026);
#2299=ELLIPSE('',#108010,0.146691465566891,0.127050784763883);
#2300=ELLIPSE('',#108027,0.1466928618908,0.127051669382332);
#2301=ELLIPSE('',#108038,0.146691465566753,0.127050784763768);
#2302=ELLIPSE('',#108042,0.146692861886957,0.127051669379919);
#2303=ELLIPSE('',#108054,0.146691465566667,0.127050784763711);
#2304=ELLIPSE('',#108071,0.146692861884917,0.127051669378417);
#2305=ELLIPSE('',#108082,0.146691465566951,0.127050784763875);
#2306=ELLIPSE('',#108086,0.146692861887784,0.127051669379951);
#2307=ELLIPSE('',#108098,0.146691465566662,0.127050784763678);
#2308=ELLIPSE('',#108115,0.146692861892035,0.127051669382384);
#2309=ELLIPSE('',#108126,0.146691465567551,0.127050784764446);
#2310=ELLIPSE('',#108130,0.146692861887898,0.127051669378866);
#2311=ELLIPSE('',#108142,0.146691465567286,0.127050784764234);
#2312=ELLIPSE('',#108159,0.146692861889581,0.127051669381123);
#2313=ELLIPSE('',#108170,0.146691465566912,0.127050784763782);
#2314=ELLIPSE('',#108174,0.146692861886619,0.127051669379193);
#2315=ELLIPSE('',#108186,0.146691465566984,0.127050784763962);
#2316=ELLIPSE('',#108203,0.14669286188925,0.127051669380939);
#2317=ELLIPSE('',#108214,0.146691465567033,0.127050784764007);
#2318=ELLIPSE('',#108218,0.146692861889623,0.127051669381043);
#2319=ELLIPSE('',#108230,0.14669146556684,0.127050784763757);
#2320=ELLIPSE('',#108247,0.146692861888148,0.127051669379703);
#2321=ELLIPSE('',#108258,0.146691465566664,0.127050784763589);
#2322=ELLIPSE('',#108262,0.146692861888369,0.127051669379955);
#2323=ELLIPSE('',#108274,0.146691465566977,0.127050784763914);
#2324=ELLIPSE('',#108291,0.146692861889199,0.127051669380361);
#2325=ELLIPSE('',#108302,0.146691465567016,0.127050784763939);
#2326=ELLIPSE('',#108306,0.146692861888996,0.127051669380984);
#2327=ELLIPSE('',#108318,0.146691465567128,0.127050784764104);
#2328=ELLIPSE('',#108335,0.146692861888997,0.127051669381534);
#2329=ELLIPSE('',#108346,0.146691465567221,0.127050784764197);
#2330=ELLIPSE('',#108350,0.146692861885338,0.12705166937903);
#2331=ELLIPSE('',#108362,0.146691465566555,0.127050784763588);
#2332=ELLIPSE('',#108379,0.146692861886485,0.127051669379774);
#2333=ELLIPSE('',#108390,0.146691465567292,0.127050784764165);
#2334=ELLIPSE('',#108394,0.146692861889409,0.12705166938008);
#2335=ELLIPSE('',#108406,0.146691465567198,0.127050784764133);
#2336=ELLIPSE('',#108423,0.146692861888131,0.127051669379491);
#2337=ELLIPSE('',#108434,0.146691465567096,0.127050784764072);
#2338=ELLIPSE('',#108438,0.146692861890808,0.127051669382308);
#2339=ELLIPSE('',#108450,0.146691465566607,0.127050784763588);
#2340=ELLIPSE('',#108467,0.146692861888626,0.127051669381254);
#2341=ELLIPSE('',#108478,0.1466914655668,0.127050784763833);
#2342=ELLIPSE('',#108482,0.146692861887797,0.127051669379309);
#2343=ELLIPSE('',#108494,0.146691465567039,0.127050784763956);
#2344=ELLIPSE('',#108511,0.146692861888548,0.127051669380616);
#2345=ELLIPSE('',#108522,0.146691465567481,0.127050784764359);
#2346=ELLIPSE('',#108526,0.146692861889464,0.127051669380601);
#2347=ELLIPSE('',#108538,0.146691465567513,0.12705078476439);
#2348=ELLIPSE('',#108555,0.146692861889216,0.127051669380696);
#2349=ELLIPSE('',#108566,0.146691465566864,0.127050784763858);
#2350=ELLIPSE('',#108570,0.146692861885317,0.127051669379159);
#2351=ELLIPSE('',#108582,0.146691465566895,0.127050784763869);
#2352=ELLIPSE('',#108599,0.146692861887918,0.127051669380084);
#2353=ELLIPSE('',#108610,0.146691465568625,0.127050784765417);
#2354=ELLIPSE('',#108614,0.146692861887782,0.127051669379891);
#2355=ELLIPSE('',#108626,0.146691465567337,0.127050784764302);
#2356=ELLIPSE('',#108643,0.146692861890565,0.127051669381493);
#2357=ELLIPSE('',#108654,0.146691465567523,0.127050784764429);
#2358=ELLIPSE('',#108658,0.146692861890385,0.127051669380385);
#2359=ELLIPSE('',#108670,0.14669146556753,0.127050784764438);
#2360=ELLIPSE('',#108687,0.146692861885322,0.127051669378044);
#2361=ELLIPSE('',#108698,0.146691465567394,0.127050784764246);
#2362=ELLIPSE('',#108702,0.146692861888362,0.127051669380383);
#2363=ELLIPSE('',#108714,0.146691465566958,0.127050784763904);
#2364=ELLIPSE('',#108731,0.146692861887648,0.12705166938048);
#2365=ELLIPSE('',#108742,0.146691465567457,0.127050784764309);
#2366=ELLIPSE('',#108746,0.14669286188913,0.127051669379752);
#2367=ELLIPSE('',#108758,0.146691465567296,0.127050784764243);
#2368=ELLIPSE('',#108775,0.146692861888268,0.127051669379853);
#2369=ELLIPSE('',#108786,0.146691465567949,0.127050784764882);
#2370=ELLIPSE('',#108790,0.146692861887034,0.12705166937996);
#2371=ELLIPSE('',#108802,0.146691465566988,0.127050784763918);
#2372=ELLIPSE('',#108819,0.14669286188752,0.127051669380341);
#2373=ELLIPSE('',#108830,0.146691465567924,0.12705078476488);
#2374=ELLIPSE('',#108834,0.146692861887905,0.127051669379344);
#2375=ELLIPSE('',#108846,0.146691465566944,0.127050784763925);
#2376=ELLIPSE('',#108863,0.146692861887371,0.127051669379764);
#2377=ELLIPSE('',#108874,0.146691465566594,0.127050784763522);
#2378=ELLIPSE('',#108878,0.146692861889815,0.127051669381089);
#2379=ELLIPSE('',#108890,0.146691465567249,0.12705078476415);
#2380=ELLIPSE('',#108901,0.146692861890005,0.127051669381267);
#2381=ELLIPSE('',#108912,0.146691465567655,0.12705078476452);
#2382=ELLIPSE('',#108916,0.1466928618887,0.127051669381071);
#2383=ELLIPSE('',#108928,0.146691465566767,0.127050784763724);
#2384=ELLIPSE('',#108945,0.146692861888402,0.127051669379751);
#2385=ELLIPSE('',#108956,0.146691465567649,0.127050784764565);
#2386=ELLIPSE('',#108960,0.146692861888125,0.127051669380703);
#2387=ELLIPSE('',#108972,0.146691465567162,0.127050784764084);
#2388=ELLIPSE('',#108989,0.146692861887572,0.127051669379447);
#2389=ELLIPSE('',#109000,0.146691465566936,0.127050784763924);
#2390=ELLIPSE('',#109004,0.146692861886526,0.127051669379105);
#2391=ELLIPSE('',#109016,0.146691465567167,0.127050784764051);
#2392=ELLIPSE('',#109033,0.146692861888572,0.127051669380327);
#2393=ELLIPSE('',#109044,0.146691465567357,0.127050784764316);
#2394=ELLIPSE('',#109048,0.146692861887322,0.127051669379629);
#2395=ELLIPSE('',#109060,0.146691465567351,0.127050784764243);
#2396=ELLIPSE('',#109077,0.146692861887703,0.127051669380563);
#2397=ELLIPSE('',#109088,0.146691465566607,0.127050784763618);
#2398=ELLIPSE('',#109092,0.146692861885829,0.127051669379383);
#2399=ELLIPSE('',#109104,0.14669146556753,0.127050784764348);
#2400=ELLIPSE('',#109121,0.14669286188798,0.127051669380014);
#2401=ELLIPSE('',#109132,0.146691465566935,0.127050784763918);
#2402=ELLIPSE('',#109136,0.146692861886356,0.127051669379263);
#2403=ELLIPSE('',#109148,0.146691465566887,0.127050784763808);
#2404=ELLIPSE('',#109165,0.146692861885907,0.127051669379342);
#2405=ELLIPSE('',#109176,0.146691465567757,0.127050784764672);
#2406=ELLIPSE('',#109180,0.146692861884678,0.12705166937695);
#2407=ELLIPSE('',#109192,0.146691465567185,0.127050784764166);
#2408=ELLIPSE('',#109209,0.146692861890572,0.127051669381342);
#2409=ELLIPSE('',#109220,0.146691465567066,0.127050784764021);
#2410=ELLIPSE('',#109224,0.146692861888206,0.12705166937956);
#2411=ELLIPSE('',#109236,0.146691465566877,0.127050784763825);
#2412=ELLIPSE('',#109253,0.146692861887242,0.127051669379058);
#2413=ELLIPSE('',#109264,0.146691465568348,0.127050784765209);
#2414=ELLIPSE('',#109268,0.146692861888642,0.127051669380438);
#2415=ELLIPSE('',#109280,0.146691465566805,0.127050784763759);
#2416=ELLIPSE('',#109297,0.146692861889443,0.127051669380692);
#2417=ELLIPSE('',#109308,0.146691465567603,0.127050784764421);
#2418=ELLIPSE('',#109312,0.146692861887422,0.127051669380312);
#2419=ELLIPSE('',#109324,0.14669146556689,0.127050784763862);
#2420=ELLIPSE('',#109341,0.146692861889481,0.127051669381202);
#2421=ELLIPSE('',#109352,0.1466914655671,0.127050784763995);
#2422=ELLIPSE('',#109356,0.146692861887204,0.127051669379616);
#2423=ELLIPSE('',#109368,0.146691465567273,0.127050784764272);
#2424=ELLIPSE('',#109385,0.146692861888368,0.127051669380196);
#2425=ELLIPSE('',#109396,0.146691465567354,0.127050784764149);
#2426=ELLIPSE('',#109400,0.146692861890029,0.127051669381068);
#2427=ELLIPSE('',#109412,0.146691465567345,0.127050784764251);
#2428=ELLIPSE('',#109429,0.146692861886787,0.127051669379225);
#2429=ELLIPSE('',#109440,0.14669146556616,0.127050784763233);
#2430=ELLIPSE('',#109444,0.146692861890226,0.127051669380676);
#2431=ELLIPSE('',#109456,0.146691465567008,0.127050784763999);
#2432=ELLIPSE('',#109473,0.146692861888184,0.127051669380381);
#2433=ELLIPSE('',#109484,0.146691465566748,0.127050784763769);
#2434=ELLIPSE('',#109488,0.146692861885311,0.127051669377263);
#2435=ELLIPSE('',#109500,0.146691465566819,0.127050784763813);
#2436=ELLIPSE('',#109517,0.146692861886789,0.127051669379176);
#2437=ELLIPSE('',#109528,0.146691465567026,0.127050784764011);
#2438=ELLIPSE('',#109532,0.146692861886493,0.127051669378802);
#2439=ELLIPSE('',#109544,0.146691465566968,0.127050784763933);
#2440=ELLIPSE('',#109555,0.146692861884915,0.127051669378065);
#2441=ELLIPSE('',#109566,0.146691465567284,0.127050784764167);
#2442=ELLIPSE('',#109570,0.146692861887552,0.127051669379605);
#2443=ELLIPSE('',#109582,0.146691465567139,0.127050784764066);
#2444=ELLIPSE('',#109599,0.146692861886816,0.12705166937847);
#2445=ELLIPSE('',#109610,0.1466914655673,0.127050784764209);
#2446=ELLIPSE('',#109614,0.146692861889501,0.127051669381896);
#2447=ELLIPSE('',#109626,0.146691465566451,0.127050784763435);
#2448=ELLIPSE('',#109643,0.146692861887066,0.127051669379779);
#2449=ELLIPSE('',#109654,0.14669146556654,0.127050784763608);
#2450=ELLIPSE('',#109658,0.146692861888615,0.12705166938038);
#2451=ELLIPSE('',#109670,0.146691465567071,0.127050784764075);
#2452=ELLIPSE('',#109687,0.146692861887632,0.127051669379309);
#2453=ELLIPSE('',#109698,0.146691465566808,0.127050784763736);
#2454=ELLIPSE('',#109702,0.146692861884796,0.127051669377432);
#2455=ELLIPSE('',#109714,0.146691465567388,0.127050784764305);
#2456=ELLIPSE('',#109731,0.146692861888991,0.127051669380517);
#2457=ELLIPSE('',#109742,0.146691465566864,0.127050784763845);
#2458=ELLIPSE('',#109746,0.146692861884702,0.127051669377471);
#2459=ELLIPSE('',#109758,0.146691465566428,0.127050784763449);
#2460=ELLIPSE('',#109775,0.146692861890953,0.127051669380815);
#2461=ELLIPSE('',#109786,0.146691465567053,0.127050784764001);
#2462=ELLIPSE('',#109790,0.146692861888345,0.1270516693799);
#2463=ELLIPSE('',#109802,0.146691465567222,0.12705078476413);
#2464=ELLIPSE('',#109819,0.146692861888203,0.127051669381085);
#2465=ELLIPSE('',#109830,0.146691465566776,0.12705078476376);
#2466=ELLIPSE('',#109834,0.146692861887467,0.127051669379034);
#2467=ELLIPSE('',#109846,0.14669146556693,0.127050784763931);
#2468=ELLIPSE('',#109863,0.146692861889339,0.127051669380069);
#2469=ELLIPSE('',#109874,0.146691465567031,0.127050784764045);
#2470=ELLIPSE('',#109878,0.146692861888236,0.127051669380494);
#2471=ELLIPSE('',#109890,0.146691465566649,0.127050784763597);
#2472=ELLIPSE('',#109907,0.146692861886606,0.127051669379421);
#2473=ELLIPSE('',#109918,0.14669146556708,0.127050784763953);
#2474=ELLIPSE('',#109922,0.146692861889654,0.127051669380473);
#2475=ELLIPSE('',#109934,0.146691465567106,0.127050784764044);
#2476=ELLIPSE('',#109951,0.146692861882192,0.127051669376308);
#2477=ELLIPSE('',#109962,0.14669146556671,0.127050784763768);
#2478=ELLIPSE('',#109966,0.146692861888881,0.127051669380729);
#2479=ELLIPSE('',#109978,0.14669146556744,0.127050784764356);
#2480=ELLIPSE('',#109995,0.146692861881194,0.127051669375846);
#2481=ELLIPSE('',#110006,0.146691465567076,0.127050784764015);
#2482=ELLIPSE('',#110010,0.146692861885841,0.127051669378297);
#2483=ELLIPSE('',#110022,0.146691465566904,0.127050784763881);
#2484=ELLIPSE('',#110039,0.146692861885695,0.127051669379351);
#2485=ELLIPSE('',#110050,0.146691465567641,0.12705078476453);
#2486=ELLIPSE('',#110054,0.146692861885858,0.127051669378641);
#2487=ELLIPSE('',#110066,0.146691465566973,0.127050784763915);
#2488=ELLIPSE('',#110083,0.146692861889958,0.127051669381835);
#2489=ELLIPSE('',#110094,0.146691465567342,0.127050784764266);
#2490=ELLIPSE('',#110098,0.146692861885233,0.127051669378449);
#2491=ELLIPSE('',#110110,0.146691465566801,0.127050784763771);
#2492=ELLIPSE('',#110127,0.14669286188867,0.127051669380722);
#2493=ELLIPSE('',#110138,0.146691465567151,0.127050784764096);
#2494=ELLIPSE('',#110142,0.146692861885986,0.127051669378141);
#2495=ELLIPSE('',#110154,0.14669146556678,0.127050784763731);
#2496=ELLIPSE('',#110171,0.146692861887676,0.127051669379299);
#2497=ELLIPSE('',#110182,0.146691465566652,0.127050784763613);
#2498=ELLIPSE('',#110386,11.6598168140706,6.11693208644189);
#2499=ELLIPSE('',#110472,1.76555576320667,1.39650815276582);
#2500=ELLIPSE('',#110588,4.72274651081773,4.72274160816237);
#2506=(
BOUNDED_SURFACE()
B_SPLINE_SURFACE(3,2,((#182277,#182278,#182279),(#182280,#182281,#182282),
(#182283,#182284,#182285),(#182286,#182287,#182288)),.UNSPECIFIED.,.F.,
 .F.,.F.)
B_SPLINE_SURFACE_WITH_KNOTS((4,4),(3,3),(0.,0.000397394410828739),(0.,1.),
 .UNSPECIFIED.)
GEOMETRIC_REPRESENTATION_ITEM()
RATIONAL_B_SPLINE_SURFACE(((1.,0.708689770883314,1.),(1.,0.708376440034512,
1.),(1.,0.707750498698405,1.),(1.,0.707106781186548,1.)))
REPRESENTATION_ITEM('')
SURFACE()
);
#2507=(
BOUNDED_SURFACE()
B_SPLINE_SURFACE(3,2,((#182294,#182295,#182296),(#182297,#182298,#182299),
(#182300,#182301,#182302),(#182303,#182304,#182305)),.UNSPECIFIED.,.F.,
 .F.,.F.)
B_SPLINE_SURFACE_WITH_KNOTS((4,4),(3,3),(0.,0.000511815090126176),(0.,1.00105592270548),
 .UNSPECIFIED.)
GEOMETRIC_REPRESENTATION_ITEM()
RATIONAL_B_SPLINE_SURFACE(((1.,0.70526624271652,1.00062243213277),(1.,0.705584085908178,
1.00062176089709),(1.,0.706182089449526,1.00062049800605),(1.,0.706797508586522,
1.00061919833597)))
REPRESENTATION_ITEM('')
SURFACE()
);
#2508=(
BOUNDED_SURFACE()
B_SPLINE_SURFACE(3,2,((#182307,#182308,#182309),(#182310,#182311,#182312),
(#182313,#182314,#182315),(#182316,#182317,#182318)),.UNSPECIFIED.,.F.,
 .F.,.F.)
B_SPLINE_SURFACE_WITH_KNOTS((4,4),(3,3),(-6.85757874097082E-18,0.000397394428086617),
(0.,1.),.UNSPECIFIED.)
GEOMETRIC_REPRESENTATION_ITEM()
RATIONAL_B_SPLINE_SURFACE(((1.,0.707106781186548,1.),(1.,0.706459846759102,
1.),(1.,0.705820510737261,1.),(1.,0.705498956110752,1.)))
REPRESENTATION_ITEM('')
SURFACE()
);
#2509=(
BOUNDED_SURFACE()
B_SPLINE_SURFACE(3,2,((#182324,#182325,#182326),(#182327,#182328,#182329),
(#182330,#182331,#182332),(#182333,#182334,#182335),(#182336,#182337,#182338),
(#182339,#182340,#182341)),.UNSPECIFIED.,.F.,.F.,.F.)
B_SPLINE_SURFACE_WITH_KNOTS((4,2,4),(3,3),(0.,0.000257953807872846,0.000515907615745692),
(0.,1.),.UNSPECIFIED.)
GEOMETRIC_REPRESENTATION_ITEM()
RATIONAL_B_SPLINE_SURFACE(((1.,0.874619707139392,1.),(1.,0.874834349678941,
1.),(1.,0.854686104157853,1.),(1.,0.792476597915084,1.),(1.,0.750887854595174,
1.),(1.,0.705585838031441,1.)))
REPRESENTATION_ITEM('')
SURFACE()
);
#2510=(
BOUNDED_SURFACE()
B_SPLINE_SURFACE(3,2,((#182347,#182348,#182349),(#182350,#182351,#182352),
(#182353,#182354,#182355),(#182356,#182357,#182358)),.UNSPECIFIED.,.F.,
 .F.,.F.)
B_SPLINE_SURFACE_WITH_KNOTS((4,4),(3,3),(0.,0.000511815437699147),(0.,1.00105881331497),
 .UNSPECIFIED.)
GEOMETRIC_REPRESENTATION_ITEM()
RATIONAL_B_SPLINE_SURFACE(((1.,0.706796661946604,1.00062089519665),(1.,
0.707430821225471,1.00061955228407),(1.,0.708058545830999,1.00061822299773),
(1.,0.708394505252984,1.00061751156111)))
REPRESENTATION_ITEM('')
SURFACE()
);
#2511=(
BOUNDED_SURFACE()
B_SPLINE_SURFACE(3,2,((#182360,#182361,#182362),(#182363,#182364,#182365),
(#182366,#182367,#182368),(#182369,#182370,#182371),(#182372,#182373,#182374),
(#182375,#182376,#182377)),.UNSPECIFIED.,.F.,.F.,.F.)
B_SPLINE_SURFACE_WITH_KNOTS((4,2,4),(3,3),(0.,0.000256915317531259,0.000513830635062519),
(0.,1.),.UNSPECIFIED.)
GEOMETRIC_REPRESENTATION_ITEM()
RATIONAL_B_SPLINE_SURFACE(((1.,0.705585838031441,1.),(1.,0.750902433542908,
1.),(1.,0.7923295300823,1.),(1.,0.854288401594408,1.),(1.,0.874998031124972,
1.),(1.,0.874619707139392,1.)))
REPRESENTATION_ITEM('')
SURFACE()
);
#2512=(
BOUNDED_SURFACE()
B_SPLINE_SURFACE(3,2,((#182383,#182384,#182385),(#182386,#182387,#182388),
(#182389,#182390,#182391),(#182392,#182393,#182394),(#182395,#182396,#182397),
(#182398,#182399,#182400)),.UNSPECIFIED.,.F.,.F.,.F.)
B_SPLINE_SURFACE_WITH_KNOTS((4,2,4),(3,3),(-1.35525271560688E-19,0.000256592814262156,
0.000513185628524312),(0.,1.),.UNSPECIFIED.)
GEOMETRIC_REPRESENTATION_ITEM()
RATIONAL_B_SPLINE_SURFACE(((1.,0.708712527163663,1.),(1.,0.753780902613751,
1.),(1.,0.794538995768995,1.),(1.,0.855070770331318,1.),(1.,0.875018427445164,
1.),(1.,0.874619707139396,1.)))
REPRESENTATION_ITEM('')
SURFACE()
);
#2513=(
BOUNDED_SURFACE()
B_SPLINE_SURFACE(3,2,((#182402,#182403,#182404),(#182405,#182406,#182407),
(#182408,#182409,#182410),(#182411,#182412,#182413)),.UNSPECIFIED.,.F.,
 .F.,.F.)
B_SPLINE_SURFACE_WITH_KNOTS((4,4),(3,3),(2.71050543121376E-20,0.000511815072430401),
(0.,1.00105598366171),.UNSPECIFIED.)
GEOMETRIC_REPRESENTATION_ITEM()
RATIONAL_B_SPLINE_SURFACE(((1.,0.706797490732854,1.00061923411872),(1.,
0.706182062145767,1.00062053388378),(1.,0.705584062768141,1.00062179683893),
(1.,0.70526622476961,1.0006224681024)))
REPRESENTATION_ITEM('')
SURFACE()
);
#2514=(
BOUNDED_SURFACE()
B_SPLINE_SURFACE(3,2,((#182419,#182420,#182421),(#182422,#182423,#182424),
(#182425,#182426,#182427),(#182428,#182429,#182430),(#182431,#182432,#182433),
(#182434,#182435,#182436)),.UNSPECIFIED.,.F.,.F.,.F.)
B_SPLINE_SURFACE_WITH_KNOTS((4,2,4),(3,3),(0.,0.000257652232350879,0.000515304464701757),
(0.,1.),.UNSPECIFIED.)
GEOMETRIC_REPRESENTATION_ITEM()
RATIONAL_B_SPLINE_SURFACE(((1.,0.87461970713939,1.),(1.,0.874861180430742,
1.),(1.,0.855455725920812,1.),(1.,0.794699358955327,1.),(1.,0.753768977788612,
1.),(1.,0.708712527163663,1.)))
REPRESENTATION_ITEM('')
SURFACE()
);
#2515=(
BOUNDED_SURFACE()
B_SPLINE_SURFACE(3,2,((#182442,#182443,#182444),(#182445,#182446,#182447),
(#182448,#182449,#182450),(#182451,#182452,#182453)),.UNSPECIFIED.,.F.,
 .F.,.F.)
B_SPLINE_SURFACE_WITH_KNOTS((4,4),(3,3),(0.,0.000397394373651911),(0.,1.),
 .UNSPECIFIED.)
GEOMETRIC_REPRESENTATION_ITEM()
RATIONAL_B_SPLINE_SURFACE(((1.,0.707106781186548,1.),(1.,0.707752587915878,
1.),(1.,0.708377654540693,1.),(1.,0.708689770883314,1.)))
REPRESENTATION_ITEM('')
SURFACE()
);
#2516=(
BOUNDED_SURFACE()
B_SPLINE_SURFACE(3,2,((#182455,#182456,#182457),(#182458,#182459,#182460),
(#182461,#182462,#182463),(#182464,#182465,#182466)),.UNSPECIFIED.,.F.,
 .F.,.F.)
B_SPLINE_SURFACE_WITH_KNOTS((4,4),(3,3),(-6.42389787197661E-18,0.000511815456479793),
(0.,1.00105873159743),.UNSPECIFIED.)
GEOMETRIC_REPRESENTATION_ITEM()
RATIONAL_B_SPLINE_SURFACE(((1.,0.70839452905708,1.00061746385214),(1.,0.708058564167607,
1.00061817524543),(1.,0.707430835372803,1.00061950443805),(1.,0.706796685881118,
1.00062084722626)))
REPRESENTATION_ITEM('')
SURFACE()
);
#2517=(
BOUNDED_SURFACE()
B_SPLINE_SURFACE(3,2,((#182472,#182473,#182474),(#182475,#182476,#182477),
(#182478,#182479,#182480),(#182481,#182482,#182483)),.UNSPECIFIED.,.F.,
 .F.,.F.)
B_SPLINE_SURFACE_WITH_KNOTS((4,4),(3,3),(0.,0.000397394465448317),(0.,1.),
 .UNSPECIFIED.)
GEOMETRIC_REPRESENTATION_ITEM()
RATIONAL_B_SPLINE_SURFACE(((1.,0.705498956110752,1.),(1.,0.705821764811793,
1.),(1.,0.70646195252114,1.),(1.,0.707106781186548,1.)))
REPRESENTATION_ITEM('')
SURFACE()
);
#2518=(
BOUNDED_SURFACE()
B_SPLINE_SURFACE(3,2,((#197994,#197995,#197996),(#197997,#197998,#197999),
(#198000,#198001,#198002),(#198003,#198004,#198005)),.UNSPECIFIED.,.F.,
 .F.,.F.)
B_SPLINE_SURFACE_WITH_KNOTS((4,4),(3,3),(0.,0.000397394410828745),(0.,1.),
 .UNSPECIFIED.)
GEOMETRIC_REPRESENTATION_ITEM()
RATIONAL_B_SPLINE_SURFACE(((1.,0.708689770883337,1.),(1.,0.708376440034498,
1.),(1.,0.707750498698412,1.),(1.,0.707106781186545,1.)))
REPRESENTATION_ITEM('')
SURFACE()
);
#2519=(
BOUNDED_SURFACE()
B_SPLINE_SURFACE(3,2,((#198011,#198012,#198013),(#198014,#198015,#198016),
(#198017,#198018,#198019),(#198020,#198021,#198022)),.UNSPECIFIED.,.F.,
 .F.,.F.)
B_SPLINE_SURFACE_WITH_KNOTS((4,4),(3,3),(0.,0.000511815090126173),(0.,1.0010559227043),
 .UNSPECIFIED.)
GEOMETRIC_REPRESENTATION_ITEM()
RATIONAL_B_SPLINE_SURFACE(((1.,0.705266242716861,1.00062243213208),(1.,
0.705584085908513,1.00062176089639),(1.,0.706182089449887,1.00062049800536),
(1.,0.706797508586863,1.00061919833528)))
REPRESENTATION_ITEM('')
SURFACE()
);
#2520=(
BOUNDED_SURFACE()
B_SPLINE_SURFACE(3,2,((#198024,#198025,#198026),(#198027,#198028,#198029),
(#198030,#198031,#198032),(#198033,#198034,#198035)),.UNSPECIFIED.,.F.,
 .F.,.F.)
B_SPLINE_SURFACE_WITH_KNOTS((4,4),(3,3),(0.,0.000397394428086619),(0.,1.),
 .UNSPECIFIED.)
GEOMETRIC_REPRESENTATION_ITEM()
RATIONAL_B_SPLINE_SURFACE(((1.,0.70710678118655,1.),(1.,0.706459846759069,
1.),(1.,0.705820510737317,1.),(1.,0.705498956110744,1.)))
REPRESENTATION_ITEM('')
SURFACE()
);
#2521=(
BOUNDED_SURFACE()
B_SPLINE_SURFACE(3,2,((#198041,#198042,#198043),(#198044,#198045,#198046),
(#198047,#198048,#198049),(#198050,#198051,#198052),(#198053,#198054,#198055),
(#198056,#198057,#198058)),.UNSPECIFIED.,.F.,.F.,.F.)
B_SPLINE_SURFACE_WITH_KNOTS((4,2,4),(3,3),(0.,0.000257953807872849,0.000515907615745699),
(0.,1.),.UNSPECIFIED.)
GEOMETRIC_REPRESENTATION_ITEM()
RATIONAL_B_SPLINE_SURFACE(((1.,0.874619707139388,1.),(1.,0.874834349679073,
1.),(1.,0.854686104157671,1.),(1.,0.792476597915277,1.),(1.,0.750887854595045,
1.),(1.,0.705585838031441,1.)))
REPRESENTATION_ITEM('')
SURFACE()
);
#2522=(
BOUNDED_SURFACE()
B_SPLINE_SURFACE(3,2,((#198064,#198065,#198066),(#198067,#198068,#198069),
(#198070,#198071,#198072),(#198073,#198074,#198075)),.UNSPECIFIED.,.F.,
 .F.,.F.)
B_SPLINE_SURFACE_WITH_KNOTS((4,4),(3,3),(0.,0.000511815437699156),(0.,1.00105881331658),
 .UNSPECIFIED.)
GEOMETRIC_REPRESENTATION_ITEM()
RATIONAL_B_SPLINE_SURFACE(((1.,0.706796661946134,1.00062089519759),(1.,
0.707430821225006,1.00061955228502),(1.,0.708058545830511,1.00061822299867),
(1.,0.708394505252524,1.00061751156205)))
REPRESENTATION_ITEM('')
SURFACE()
);
#2523=(
BOUNDED_SURFACE()
B_SPLINE_SURFACE(3,2,((#198077,#198078,#198079),(#198080,#198081,#198082),
(#198083,#198084,#198085),(#198086,#198087,#198088),(#198089,#198090,#198091),
(#198092,#198093,#198094)),.UNSPECIFIED.,.F.,.F.,.F.)
B_SPLINE_SURFACE_WITH_KNOTS((4,2,4),(3,3),(0.,0.000256915317531264,0.000513830635062528),
(0.,1.),.UNSPECIFIED.)
GEOMETRIC_REPRESENTATION_ITEM()
RATIONAL_B_SPLINE_SURFACE(((1.,0.70558583803145,1.),(1.,0.750902433543446,
1.),(1.,0.792329530081587,1.),(1.,0.854288401595139,1.),(1.,0.874998031124452,
1.),(1.,0.874619707139387,1.)))
REPRESENTATION_ITEM('')
SURFACE()
);
#2524=(
BOUNDED_SURFACE()
B_SPLINE_SURFACE(3,2,((#198100,#198101,#198102),(#198103,#198104,#198105),
(#198106,#198107,#198108),(#198109,#198110,#198111),(#198112,#198113,#198114),
(#198115,#198116,#198117)),.UNSPECIFIED.,.F.,.F.,.F.)
B_SPLINE_SURFACE_WITH_KNOTS((4,2,4),(3,3),(0.,0.000256592814262158,0.000513185628524315),
(0.,1.),.UNSPECIFIED.)
GEOMETRIC_REPRESENTATION_ITEM()
RATIONAL_B_SPLINE_SURFACE(((1.,0.708712527163671,1.),(1.,0.753780902613744,
1.),(1.,0.794538995768995,1.),(1.,0.855070770331309,1.),(1.,0.875018427445166,
1.),(1.,0.87461970713939,1.)))
REPRESENTATION_ITEM('')
SURFACE()
);
#2525=(
BOUNDED_SURFACE()
B_SPLINE_SURFACE(3,2,((#198119,#198120,#198121),(#198122,#198123,#198124),
(#198125,#198126,#198127),(#198128,#198129,#198130)),.UNSPECIFIED.,.F.,
 .F.,.F.)
B_SPLINE_SURFACE_WITH_KNOTS((4,4),(3,3),(0.,0.000511815072430398),(0.,1.00105598365828),
 .UNSPECIFIED.)
GEOMETRIC_REPRESENTATION_ITEM()
RATIONAL_B_SPLINE_SURFACE(((1.,0.70679749073386,1.0006192341167),(1.,0.706182062146784,
1.00062053388176),(1.,0.705584062769139,1.00062179683691),(1.,0.705266224770628,
1.00062246810037)))
REPRESENTATION_ITEM('')
SURFACE()
);
#2526=(
BOUNDED_SURFACE()
B_SPLINE_SURFACE(3,2,((#198136,#198137,#198138),(#198139,#198140,#198141),
(#198142,#198143,#198144),(#198145,#198146,#198147),(#198148,#198149,#198150),
(#198151,#198152,#198153)),.UNSPECIFIED.,.F.,.F.,.F.)
B_SPLINE_SURFACE_WITH_KNOTS((4,2,4),(3,3),(1.35525271560688E-20,0.000257652232350883,
0.000515304464701766),(0.,1.),.UNSPECIFIED.)
GEOMETRIC_REPRESENTATION_ITEM()
RATIONAL_B_SPLINE_SURFACE(((1.,0.874619707139378,1.),(1.,0.874861180430966,
1.),(1.,0.855455725920513,1.),(1.,0.794699358955603,1.),(1.,0.753768977788378,
1.),(1.,0.708712527163653,1.)))
REPRESENTATION_ITEM('')
SURFACE()
);
#2527=(
BOUNDED_SURFACE()
B_SPLINE_SURFACE(3,2,((#198159,#198160,#198161),(#198162,#198163,#198164),
(#198165,#198166,#198167),(#198168,#198169,#198170)),.UNSPECIFIED.,.F.,
 .F.,.F.)
B_SPLINE_SURFACE_WITH_KNOTS((4,4),(3,3),(-2.71050543121376E-20,0.00039739437365192),
(0.,1.),.UNSPECIFIED.)
GEOMETRIC_REPRESENTATION_ITEM()
RATIONAL_B_SPLINE_SURFACE(((1.,0.707106781186548,1.),(1.,0.707752587915895,
1.),(1.,0.70837765454067,1.),(1.,0.708689770883327,1.)))
REPRESENTATION_ITEM('')
SURFACE()
);
#2528=(
BOUNDED_SURFACE()
B_SPLINE_SURFACE(3,2,((#198172,#198173,#198174),(#198175,#198176,#198177),
(#198178,#198179,#198180),(#198181,#198182,#198183)),.UNSPECIFIED.,.F.,
 .F.,.F.)
B_SPLINE_SURFACE_WITH_KNOTS((4,4),(3,3),(0.,0.000511815456479787),(0.,1.00105873159873),
 .UNSPECIFIED.)
GEOMETRIC_REPRESENTATION_ITEM()
RATIONAL_B_SPLINE_SURFACE(((1.,0.708394529056677,1.0006174638529),(1.,0.708058564167213,
1.00061817524619),(1.,0.707430835372427,1.00061950443881),(1.,0.706796685880734,
1.00062084722702)))
REPRESENTATION_ITEM('')
SURFACE()
);
#2529=(
BOUNDED_SURFACE()
B_SPLINE_SURFACE(3,2,((#198189,#198190,#198191),(#198192,#198193,#198194),
(#198195,#198196,#198197),(#198198,#198199,#198200)),.UNSPECIFIED.,.F.,
 .F.,.F.)
B_SPLINE_SURFACE_WITH_KNOTS((4,4),(3,3),(0.,0.000397394465448306),(0.,1.),
 .UNSPECIFIED.)
GEOMETRIC_REPRESENTATION_ITEM()
RATIONAL_B_SPLINE_SURFACE(((1.,0.70549895611076,1.),(1.,0.705821764811791,
1.),(1.,0.70646195252114,1.),(1.,0.707106781186548,1.)))
REPRESENTATION_ITEM('')
SURFACE()
);
#2530=(
BOUNDED_SURFACE()
B_SPLINE_SURFACE(3,2,((#198206,#198207,#198208),(#198209,#198210,#198211),
(#198212,#198213,#198214),(#198215,#198216,#198217)),.UNSPECIFIED.,.F.,
 .F.,.F.)
B_SPLINE_SURFACE_WITH_KNOTS((4,4),(3,3),(0.,0.000397394410828732),(0.,1.),
 .UNSPECIFIED.)
GEOMETRIC_REPRESENTATION_ITEM()
RATIONAL_B_SPLINE_SURFACE(((1.,0.70868977088332,1.),(1.,0.708376440034513,
1.),(1.,0.707750498698404,1.),(1.,0.707106781186548,1.)))
REPRESENTATION_ITEM('')
SURFACE()
);
#2531=(
BOUNDED_SURFACE()
B_SPLINE_SURFACE(3,2,((#198223,#198224,#198225),(#198226,#198227,#198228),
(#198229,#198230,#198231),(#198232,#198233,#198234)),.UNSPECIFIED.,.F.,
 .F.,.F.)
B_SPLINE_SURFACE_WITH_KNOTS((4,4),(3,3),(0.,0.000511815090126187),(0.,1.0010559227001),
 .UNSPECIFIED.)
GEOMETRIC_REPRESENTATION_ITEM()
RATIONAL_B_SPLINE_SURFACE(((1.,0.705266242718086,1.0006224321296),(1.,0.705584085909768,
1.00062176089392),(1.,0.706182089451109,1.00062049800289),(1.,0.706797508588093,
1.00061919833282)))
REPRESENTATION_ITEM('')
SURFACE()
);
#2532=(
BOUNDED_SURFACE()
B_SPLINE_SURFACE(3,2,((#198236,#198237,#198238),(#198239,#198240,#198241),
(#198242,#198243,#198244),(#198245,#198246,#198247)),.UNSPECIFIED.,.F.,
 .F.,.F.)
B_SPLINE_SURFACE_WITH_KNOTS((4,4),(3,3),(0.,0.000397394428086622),(0.,1.),
 .UNSPECIFIED.)
GEOMETRIC_REPRESENTATION_ITEM()
RATIONAL_B_SPLINE_SURFACE(((1.,0.707106781186544,1.),(1.,0.706459846759088,
1.),(1.,0.705820510737285,1.),(1.,0.70549895611075,1.)))
REPRESENTATION_ITEM('')
SURFACE()
);
#2533=(
BOUNDED_SURFACE()
B_SPLINE_SURFACE(3,2,((#198253,#198254,#198255),(#198256,#198257,#198258),
(#198259,#198260,#198261),(#198262,#198263,#198264),(#198265,#198266,#198267),
(#198268,#198269,#198270)),.UNSPECIFIED.,.F.,.F.,.F.)
B_SPLINE_SURFACE_WITH_KNOTS((4,2,4),(3,3),(0.,0.000257953807872845,0.000515907615745691),
(0.,1.),.UNSPECIFIED.)
GEOMETRIC_REPRESENTATION_ITEM()
RATIONAL_B_SPLINE_SURFACE(((1.,0.874619707139393,1.),(1.,0.874834349679163,
1.),(1.,0.854686104157555,1.),(1.,0.792476597915392,1.),(1.,0.750887854594916,
1.),(1.,0.705585838031459,1.)))
REPRESENTATION_ITEM('')
SURFACE()
);
#2534=(
BOUNDED_SURFACE()
B_SPLINE_SURFACE(3,2,((#198276,#198277,#198278),(#198279,#198280,#198281),
(#198282,#198283,#198284),(#198285,#198286,#198287)),.UNSPECIFIED.,.F.,
 .F.,.F.)
B_SPLINE_SURFACE_WITH_KNOTS((4,4),(3,3),(0.,0.000511815437699162),(0.,1.00105881331787),
 .UNSPECIFIED.)
GEOMETRIC_REPRESENTATION_ITEM()
RATIONAL_B_SPLINE_SURFACE(((1.,0.706796661945754,1.00062089519835),(1.,
0.707430821224618,1.00061955228577),(1.,0.708058545830163,1.00061822299943),
(1.,0.70839450525214,1.00061751156281)))
REPRESENTATION_ITEM('')
SURFACE()
);
#2535=(
BOUNDED_SURFACE()
B_SPLINE_SURFACE(3,2,((#198289,#198290,#198291),(#198292,#198293,#198294),
(#198295,#198296,#198297),(#198298,#198299,#198300),(#198301,#198302,#198303),
(#198304,#198305,#198306)),.UNSPECIFIED.,.F.,.F.,.F.)
B_SPLINE_SURFACE_WITH_KNOTS((4,2,4),(3,3),(0.,0.000256915317531265,0.000513830635062529),
(0.,1.),.UNSPECIFIED.)
GEOMETRIC_REPRESENTATION_ITEM()
RATIONAL_B_SPLINE_SURFACE(((1.,0.705585838031458,1.),(1.,0.750902433542261,
1.),(1.,0.792329530083196,1.),(1.,0.854288401593537,1.),(1.,0.874998031125653,
1.),(1.,0.87461970713941,1.)))
REPRESENTATION_ITEM('')
SURFACE()
);
#2536=(
BOUNDED_SURFACE()
B_SPLINE_SURFACE(3,2,((#198312,#198313,#198314),(#198315,#198316,#198317),
(#198318,#198319,#198320),(#198321,#198322,#198323),(#198324,#198325,#198326),
(#198327,#198328,#198329)),.UNSPECIFIED.,.F.,.F.,.F.)
B_SPLINE_SURFACE_WITH_KNOTS((4,2,4),(3,3),(0.,0.000256592814262157,0.000513185628524314),
(0.,1.),.UNSPECIFIED.)
GEOMETRIC_REPRESENTATION_ITEM()
RATIONAL_B_SPLINE_SURFACE(((1.,0.708712527163673,1.),(1.,0.753780902613744,
1.),(1.,0.794538995768969,1.),(1.,0.855070770331331,1.),(1.,0.875018427445154,
1.),(1.,0.874619707139393,1.)))
REPRESENTATION_ITEM('')
SURFACE()
);
#2537=(
BOUNDED_SURFACE()
B_SPLINE_SURFACE(3,2,((#198331,#198332,#198333),(#198334,#198335,#198336),
(#198337,#198338,#198339),(#198340,#198341,#198342)),.UNSPECIFIED.,.F.,
 .F.,.F.)
B_SPLINE_SURFACE_WITH_KNOTS((4,4),(3,3),(0.,0.000511815072430393),(0.,1.00105598365973),
 .UNSPECIFIED.)
GEOMETRIC_REPRESENTATION_ITEM()
RATIONAL_B_SPLINE_SURFACE(((1.,0.706797490733436,1.00061923411755),(1.,
0.706182062146356,1.00062053388262),(1.,0.705584062768711,1.00062179683776),
(1.,0.7052662247702,1.00062246810122)))
REPRESENTATION_ITEM('')
SURFACE()
);
#2538=(
BOUNDED_SURFACE()
B_SPLINE_SURFACE(3,2,((#198348,#198349,#198350),(#198351,#198352,#198353),
(#198354,#198355,#198356),(#198357,#198358,#198359),(#198360,#198361,#198362),
(#198363,#198364,#198365)),.UNSPECIFIED.,.F.,.F.,.F.)
B_SPLINE_SURFACE_WITH_KNOTS((4,2,4),(3,3),(-1.70761842166467E-18,0.000257652232350888,
0.000515304464701778),(0.,1.),.UNSPECIFIED.)
GEOMETRIC_REPRESENTATION_ITEM()
RATIONAL_B_SPLINE_SURFACE(((1.,0.874619707139376,1.),(1.,0.874861180430913,
1.),(1.,0.85545572592056,1.),(1.,0.794699358955552,1.),(1.,0.753768977788407,
1.),(1.,0.708712527163644,1.)))
REPRESENTATION_ITEM('')
SURFACE()
);
#2539=(
BOUNDED_SURFACE()
B_SPLINE_SURFACE(3,2,((#198371,#198372,#198373),(#198374,#198375,#198376),
(#198377,#198378,#198379),(#198380,#198381,#198382)),.UNSPECIFIED.,.F.,
 .F.,.F.)
B_SPLINE_SURFACE_WITH_KNOTS((4,4),(3,3),(-7.04731412115578E-18,0.000397394373651905),
(0.,1.),.UNSPECIFIED.)
GEOMETRIC_REPRESENTATION_ITEM()
RATIONAL_B_SPLINE_SURFACE(((1.,0.707106781186542,1.),(1.,0.707752587915911,
1.),(1.,0.708377654540645,1.),(1.,0.708689770883334,1.)))
REPRESENTATION_ITEM('')
SURFACE()
);
#2540=(
BOUNDED_SURFACE()
B_SPLINE_SURFACE(3,2,((#198384,#198385,#198386),(#198387,#198388,#198389),
(#198390,#198391,#198392),(#198393,#198394,#198395)),.UNSPECIFIED.,.F.,
 .F.,.F.)
B_SPLINE_SURFACE_WITH_KNOTS((4,4),(3,3),(0.,0.000511815456479787),(0.,1.00105873159852),
 .UNSPECIFIED.)
GEOMETRIC_REPRESENTATION_ITEM()
RATIONAL_B_SPLINE_SURFACE(((1.,0.708394529056741,1.00061746385278),(1.,
0.708058564167289,1.00061817524607),(1.,0.707430835372482,1.00061950443869),
(1.,0.706796685880791,1.0006208472269)))
REPRESENTATION_ITEM('')
SURFACE()
);
#2541=(
BOUNDED_SURFACE()
B_SPLINE_SURFACE(3,2,((#198401,#198402,#198403),(#198404,#198405,#198406),
(#198407,#198408,#198409),(#198410,#198411,#198412)),.UNSPECIFIED.,.F.,
 .F.,.F.)
B_SPLINE_SURFACE_WITH_KNOTS((4,4),(3,3),(0.,0.000397394465448288),(0.,1.),
 .UNSPECIFIED.)
GEOMETRIC_REPRESENTATION_ITEM()
RATIONAL_B_SPLINE_SURFACE(((1.,0.705498956110755,1.),(1.,0.705821764811768,
1.),(1.,0.706461952521147,1.),(1.,0.707106781186548,1.)))
REPRESENTATION_ITEM('')
SURFACE()
);
#2542=(
BOUNDED_SURFACE()
B_SPLINE_SURFACE(3,2,((#198418,#198419,#198420),(#198421,#198422,#198423),
(#198424,#198425,#198426),(#198427,#198428,#198429)),.UNSPECIFIED.,.F.,
 .F.,.F.)
B_SPLINE_SURFACE_WITH_KNOTS((4,4),(3,3),(0.,0.000397394410828734),(0.,1.),
 .UNSPECIFIED.)
GEOMETRIC_REPRESENTATION_ITEM()
RATIONAL_B_SPLINE_SURFACE(((1.,0.708689770883327,1.),(1.,0.708376440034476,
1.),(1.,0.707750498698407,1.),(1.,0.707106781186548,1.)))
REPRESENTATION_ITEM('')
SURFACE()
);
#2543=(
BOUNDED_SURFACE()
B_SPLINE_SURFACE(3,2,((#198435,#198436,#198437),(#198438,#198439,#198440),
(#198441,#198442,#198443),(#198444,#198445,#198446)),.UNSPECIFIED.,.F.,
 .F.,.F.)
B_SPLINE_SURFACE_WITH_KNOTS((4,4),(3,3),(0.,0.000511815090126176),(0.,1.00105592270127),
 .UNSPECIFIED.)
GEOMETRIC_REPRESENTATION_ITEM()
RATIONAL_B_SPLINE_SURFACE(((1.,0.705266242717785,1.00062243213029),(1.,
0.705584085909388,1.00062176089461),(1.,0.706182089450783,1.00062049800358),
(1.,0.706797508587755,1.0006191983335)))
REPRESENTATION_ITEM('')
SURFACE()
);
#2544=(
BOUNDED_SURFACE()
B_SPLINE_SURFACE(3,2,((#198448,#198449,#198450),(#198451,#198452,#198453),
(#198454,#198455,#198456),(#198457,#198458,#198459)),.UNSPECIFIED.,.F.,
 .F.,.F.)
B_SPLINE_SURFACE_WITH_KNOTS((4,4),(3,3),(-7.56231015308639E-18,0.000397394428086627),
(0.,1.),.UNSPECIFIED.)
GEOMETRIC_REPRESENTATION_ITEM()
RATIONAL_B_SPLINE_SURFACE(((1.,0.707106781186548,1.),(1.,0.70645984675909,
1.),(1.,0.705820510737292,1.),(1.,0.705498956110763,1.)))
REPRESENTATION_ITEM('')
SURFACE()
);
#2545=(
BOUNDED_SURFACE()
B_SPLINE_SURFACE(3,2,((#198465,#198466,#198467),(#198468,#198469,#198470),
(#198471,#198472,#198473),(#198474,#198475,#198476),(#198477,#198478,#198479),
(#198480,#198481,#198482)),.UNSPECIFIED.,.F.,.F.,.F.)
B_SPLINE_SURFACE_WITH_KNOTS((4,2,4),(3,3),(0.,0.000257953807872845,0.00051590761574569),
(0.,1.),.UNSPECIFIED.)
GEOMETRIC_REPRESENTATION_ITEM()
RATIONAL_B_SPLINE_SURFACE(((1.,0.874619707139392,1.),(1.,0.87483434967877,
1.),(1.,0.854686104158095,1.),(1.,0.792476597914846,1.),(1.,0.75088785459531,
1.),(1.,0.705585838031467,1.)))
REPRESENTATION_ITEM('')
SURFACE()
);
#2546=(
BOUNDED_SURFACE()
B_SPLINE_SURFACE(3,2,((#198488,#198489,#198490),(#198491,#198492,#198493),
(#198494,#198495,#198496),(#198497,#198498,#198499)),.UNSPECIFIED.,.F.,
 .F.,.F.)
B_SPLINE_SURFACE_WITH_KNOTS((4,4),(3,3),(-7.56231015308639E-18,0.00051181543769914),
(0.,1.00105881331445),.UNSPECIFIED.)
GEOMETRIC_REPRESENTATION_ITEM()
RATIONAL_B_SPLINE_SURFACE(((1.,0.706796661946756,1.00062089519634),(1.,
0.707430821225626,1.00061955228377),(1.,0.70805854583114,1.00061822299743),
(1.,0.708394505253128,1.00061751156081)))
REPRESENTATION_ITEM('')
SURFACE()
);
#2547=(
BOUNDED_SURFACE()
B_SPLINE_SURFACE(3,2,((#198501,#198502,#198503),(#198504,#198505,#198506),
(#198507,#198508,#198509),(#198510,#198511,#198512),(#198513,#198514,#198515),
(#198516,#198517,#198518)),.UNSPECIFIED.,.F.,.F.,.F.)
B_SPLINE_SURFACE_WITH_KNOTS((4,2,4),(3,3),(0.,0.000256915317531265,0.000513830635062529),
(0.,1.),.UNSPECIFIED.)
GEOMETRIC_REPRESENTATION_ITEM()
RATIONAL_B_SPLINE_SURFACE(((1.,0.705585838031461,1.),(1.,0.750902433542682,
1.),(1.,0.792329530082583,1.),(1.,0.854288401594147,1.),(1.,0.874998031125177,
1.),(1.,0.874619707139394,1.)))
REPRESENTATION_ITEM('')
SURFACE()
);
#2548=(
BOUNDED_SURFACE()
B_SPLINE_SURFACE(3,2,((#198524,#198525,#198526),(#198527,#198528,#198529),
(#198530,#198531,#198532),(#198533,#198534,#198535),(#198536,#198537,#198538),
(#198539,#198540,#198541)),.UNSPECIFIED.,.F.,.F.,.F.)
B_SPLINE_SURFACE_WITH_KNOTS((4,2,4),(3,3),(-9.62229428080885E-18,0.000256592814262153,
0.000513185628524316),(0.,1.),.UNSPECIFIED.)
GEOMETRIC_REPRESENTATION_ITEM()
RATIONAL_B_SPLINE_SURFACE(((1.,0.708712527163657,1.),(1.,0.753780902614083,
1.),(1.,0.794538995768547,1.),(1.,0.855070770331749,1.),(1.,0.875018427444824,
1.),(1.,0.874619707139393,1.)))
REPRESENTATION_ITEM('')
SURFACE()
);
#2549=(
BOUNDED_SURFACE()
B_SPLINE_SURFACE(3,2,((#198543,#198544,#198545),(#198546,#198547,#198548),
(#198549,#198550,#198551),(#198552,#198553,#198554)),.UNSPECIFIED.,.F.,
 .F.,.F.)
B_SPLINE_SURFACE_WITH_KNOTS((4,4),(3,3),(2.71050543121376E-20,0.000511815072430402),
(0.,1.00105598365994),.UNSPECIFIED.)
GEOMETRIC_REPRESENTATION_ITEM()
RATIONAL_B_SPLINE_SURFACE(((1.,0.706797490733375,1.00061923411768),(1.,
0.706182062146284,1.00062053388274),(1.,0.705584062768653,1.00062179683788),
(1.,0.705266224770126,1.00062246810135)))
REPRESENTATION_ITEM('')
SURFACE()
);
#2550=(
BOUNDED_SURFACE()
B_SPLINE_SURFACE(3,2,((#198560,#198561,#198562),(#198563,#198564,#198565),
(#198566,#198567,#198568),(#198569,#198570,#198571),(#198572,#198573,#198574),
(#198575,#198576,#198577)),.UNSPECIFIED.,.F.,.F.,.F.)
B_SPLINE_SURFACE_WITH_KNOTS((4,2,4),(3,3),(-3.34747420754899E-18,0.000257652232350879,
0.000515304464701762),(0.,1.),.UNSPECIFIED.)
GEOMETRIC_REPRESENTATION_ITEM()
RATIONAL_B_SPLINE_SURFACE(((1.,0.874619707139387,1.),(1.,0.874861180430757,
1.),(1.,0.855455725920779,1.),(1.,0.79469935895536,1.),(1.,0.753768977788535,
1.),(1.,0.70871252716367,1.)))
REPRESENTATION_ITEM('')
SURFACE()
);
#2551=(
BOUNDED_SURFACE()
B_SPLINE_SURFACE(3,2,((#198583,#198584,#198585),(#198586,#198587,#198588),
(#198589,#198590,#198591),(#198592,#198593,#198594)),.UNSPECIFIED.,.F.,
 .F.,.F.)
B_SPLINE_SURFACE_WITH_KNOTS((4,4),(3,3),(0.,0.000397394373651928),(0.,1.),
 .UNSPECIFIED.)
GEOMETRIC_REPRESENTATION_ITEM()
RATIONAL_B_SPLINE_SURFACE(((1.,0.707106781186542,1.),(1.,0.70775258791588,
1.),(1.,0.708377654540697,1.),(1.,0.708689770883335,1.)))
REPRESENTATION_ITEM('')
SURFACE()
);
#2552=(
BOUNDED_SURFACE()
B_SPLINE_SURFACE(3,2,((#198596,#198597,#198598),(#198599,#198600,#198601),
(#198602,#198603,#198604),(#198605,#198606,#198607)),.UNSPECIFIED.,.F.,
 .F.,.F.)
B_SPLINE_SURFACE_WITH_KNOTS((4,4),(3,3),(0.,0.000511815456479793),(0.,1.00105873159883),
 .UNSPECIFIED.)
GEOMETRIC_REPRESENTATION_ITEM()
RATIONAL_B_SPLINE_SURFACE(((1.,0.708394529056664,1.00061746385296),(1.,
0.70805856416722,1.00061817524625),(1.,0.707430835372394,1.00061950443887),
(1.,0.706796685880702,1.00062084722708)))
REPRESENTATION_ITEM('')
SURFACE()
);
#2553=(
BOUNDED_SURFACE()
B_SPLINE_SURFACE(3,2,((#198613,#198614,#198615),(#198616,#198617,#198618),
(#198619,#198620,#198621),(#198622,#198623,#198624)),.UNSPECIFIED.,.F.,
 .F.,.F.)
B_SPLINE_SURFACE_WITH_KNOTS((4,4),(3,3),(0.,0.000397394465448311),(0.,1.),
 .UNSPECIFIED.)
GEOMETRIC_REPRESENTATION_ITEM()
RATIONAL_B_SPLINE_SURFACE(((1.,0.705498956110748,1.),(1.,0.705821764811775,
1.),(1.,0.706461952521139,1.),(1.,0.707106781186553,1.)))
REPRESENTATION_ITEM('')
SURFACE()
);
#2554=(
BOUNDED_SURFACE()
B_SPLINE_SURFACE(3,2,((#198630,#198631,#198632),(#198633,#198634,#198635),
(#198636,#198637,#198638),(#198639,#198640,#198641)),.UNSPECIFIED.,.F.,
 .F.,.F.)
B_SPLINE_SURFACE_WITH_KNOTS((4,4),(3,3),(0.,0.000397394410828753),(0.,1.),
 .UNSPECIFIED.)
GEOMETRIC_REPRESENTATION_ITEM()
RATIONAL_B_SPLINE_SURFACE(((1.,0.70868977088332,1.),(1.,0.708376440034504,
1.),(1.,0.707750498698403,1.),(1.,0.707106781186555,1.)))
REPRESENTATION_ITEM('')
SURFACE()
);
#2555=(
BOUNDED_SURFACE()
B_SPLINE_SURFACE(3,2,((#198647,#198648,#198649),(#198650,#198651,#198652),
(#198653,#198654,#198655),(#198656,#198657,#198658)),.UNSPECIFIED.,.F.,
 .F.,.F.)
B_SPLINE_SURFACE_WITH_KNOTS((4,4),(3,3),(0.,0.000511815090126176),(0.,1.00105592270358),
 .UNSPECIFIED.)
GEOMETRIC_REPRESENTATION_ITEM()
RATIONAL_B_SPLINE_SURFACE(((1.,0.705266242717103,1.00062243213165),(1.,
0.705584085908695,1.00062176089597),(1.,0.706182089450119,1.00062049800494),
(1.,0.706797508587078,1.00061919833486)))
REPRESENTATION_ITEM('')
SURFACE()
);
#2556=(
BOUNDED_SURFACE()
B_SPLINE_SURFACE(3,2,((#198660,#198661,#198662),(#198663,#198664,#198665),
(#198666,#198667,#198668),(#198669,#198670,#198671)),.UNSPECIFIED.,.F.,
 .F.,.F.)
B_SPLINE_SURFACE_WITH_KNOTS((4,4),(3,3),(0.,0.000397394428086627),(0.,1.),
 .UNSPECIFIED.)
GEOMETRIC_REPRESENTATION_ITEM()
RATIONAL_B_SPLINE_SURFACE(((1.,0.707106781186548,1.),(1.,0.706459846759099,
1.),(1.,0.705820510737278,1.),(1.,0.705498956110748,1.)))
REPRESENTATION_ITEM('')
SURFACE()
);
#2557=(
BOUNDED_SURFACE()
B_SPLINE_SURFACE(3,2,((#198677,#198678,#198679),(#198680,#198681,#198682),
(#198683,#198684,#198685),(#198686,#198687,#198688),(#198689,#198690,#198691),
(#198692,#198693,#198694)),.UNSPECIFIED.,.F.,.F.,.F.)
B_SPLINE_SURFACE_WITH_KNOTS((4,2,4),(3,3),(0.,0.000257953807872848,0.000515907615745695),
(0.,1.),.UNSPECIFIED.)
GEOMETRIC_REPRESENTATION_ITEM()
RATIONAL_B_SPLINE_SURFACE(((1.,0.874619707139388,1.),(1.,0.874834349678974,
1.),(1.,0.854686104157824,1.),(1.,0.792476597915113,1.),(1.,0.750887854595142,
1.),(1.,0.70558583803144,1.)))
REPRESENTATION_ITEM('')
SURFACE()
);
#2558=(
BOUNDED_SURFACE()
B_SPLINE_SURFACE(3,2,((#198700,#198701,#198702),(#198703,#198704,#198705),
(#198706,#198707,#198708),(#198709,#198710,#198711)),.UNSPECIFIED.,.F.,
 .F.,.F.)
B_SPLINE_SURFACE_WITH_KNOTS((4,4),(3,3),(0.,0.000511815437699155),(0.,1.0010588133174),
 .UNSPECIFIED.)
GEOMETRIC_REPRESENTATION_ITEM()
RATIONAL_B_SPLINE_SURFACE(((1.,0.706796661945892,1.00062089519808),(1.,
0.707430821224748,1.0006195522855),(1.,0.708058545830306,1.00061822299915),
(1.,0.708394505252271,1.00061751156253)))
REPRESENTATION_ITEM('')
SURFACE()
);
#2559=(
BOUNDED_SURFACE()
B_SPLINE_SURFACE(3,2,((#198713,#198714,#198715),(#198716,#198717,#198718),
(#198719,#198720,#198721),(#198722,#198723,#198724),(#198725,#198726,#198727),
(#198728,#198729,#198730)),.UNSPECIFIED.,.F.,.F.,.F.)
B_SPLINE_SURFACE_WITH_KNOTS((4,2,4),(3,3),(2.71050543121376E-20,0.000256915317531262,
0.000513830635062523),(0.,1.),.UNSPECIFIED.)
GEOMETRIC_REPRESENTATION_ITEM()
RATIONAL_B_SPLINE_SURFACE(((1.,0.705585838031443,1.),(1.,0.750902433542627,
1.),(1.,0.79232953008266,1.),(1.,0.854288401594061,1.),(1.,0.874998031125236,
1.),(1.,0.874619707139394,1.)))
REPRESENTATION_ITEM('')
SURFACE()
);
#2560=(
BOUNDED_SURFACE()
B_SPLINE_SURFACE(3,2,((#198736,#198737,#198738),(#198739,#198740,#198741),
(#198742,#198743,#198744),(#198745,#198746,#198747),(#198748,#198749,#198750),
(#198751,#198752,#198753)),.UNSPECIFIED.,.F.,.F.,.F.)
B_SPLINE_SURFACE_WITH_KNOTS((4,2,4),(3,3),(0.,0.000256592814262158,0.000513185628524317),
(0.,1.),.UNSPECIFIED.)
GEOMETRIC_REPRESENTATION_ITEM()
RATIONAL_B_SPLINE_SURFACE(((1.,0.708712527163662,1.),(1.,0.753780902613367,
1.),(1.,0.794538995769507,1.),(1.,0.855070770330791,1.),(1.,0.875018427445557,
1.),(1.,0.874619707139389,1.)))
REPRESENTATION_ITEM('')
SURFACE()
);
#2561=(
BOUNDED_SURFACE()
B_SPLINE_SURFACE(3,2,((#198755,#198756,#198757),(#198758,#198759,#198760),
(#198761,#198762,#198763),(#198764,#198765,#198766)),.UNSPECIFIED.,.F.,
 .F.,.F.)
B_SPLINE_SURFACE_WITH_KNOTS((4,4),(3,3),(0.,0.000511815072430394),(0.,1.00105598365809),
 .UNSPECIFIED.)
GEOMETRIC_REPRESENTATION_ITEM()
RATIONAL_B_SPLINE_SURFACE(((1.,0.706797490733914,1.00061923411659),(1.,
0.706182062146832,1.00062053388166),(1.,0.705584062769191,1.0006217968368),
(1.,0.705266224770676,1.00062246810026)))
REPRESENTATION_ITEM('')
SURFACE()
);
#2562=(
BOUNDED_SURFACE()
B_SPLINE_SURFACE(3,2,((#198772,#198773,#198774),(#198775,#198776,#198777),
(#198778,#198779,#198780),(#198781,#198782,#198783),(#198784,#198785,#198786),
(#198787,#198788,#198789)),.UNSPECIFIED.,.F.,.F.,.F.)
B_SPLINE_SURFACE_WITH_KNOTS((4,2,4),(3,3),(1.35525271560688E-20,0.000257652232350875,
0.00051530446470175),(0.,1.),.UNSPECIFIED.)
GEOMETRIC_REPRESENTATION_ITEM()
RATIONAL_B_SPLINE_SURFACE(((1.,0.87461970713939,1.),(1.,0.874861180430533,
1.),(1.,0.855455725921098,1.),(1.,0.794699358955019,1.),(1.,0.753768977788807,
1.),(1.,0.708712527163686,1.)))
REPRESENTATION_ITEM('')
SURFACE()
);
#2563=(
BOUNDED_SURFACE()
B_SPLINE_SURFACE(3,2,((#198795,#198796,#198797),(#198798,#198799,#198800),
(#198801,#198802,#198803),(#198804,#198805,#198806)),.UNSPECIFIED.,.F.,
 .F.,.F.)
B_SPLINE_SURFACE_WITH_KNOTS((4,4),(3,3),(0.,0.000397394373651918),(0.,1.),
 .UNSPECIFIED.)
GEOMETRIC_REPRESENTATION_ITEM()
RATIONAL_B_SPLINE_SURFACE(((1.,0.707106781186539,1.),(1.,0.707752587915889,
1.),(1.,0.708377654540736,1.),(1.,0.708689770883308,1.)))
REPRESENTATION_ITEM('')
SURFACE()
);
#2564=(
BOUNDED_SURFACE()
B_SPLINE_SURFACE(3,2,((#198808,#198809,#198810),(#198811,#198812,#198813),
(#198814,#198815,#198816),(#198817,#198818,#198819)),.UNSPECIFIED.,.F.,
 .F.,.F.)
B_SPLINE_SURFACE_WITH_KNOTS((4,4),(3,3),(0.,0.000511815456479787),(0.,1.00105873159994),
 .UNSPECIFIED.)
GEOMETRIC_REPRESENTATION_ITEM()
RATIONAL_B_SPLINE_SURFACE(((1.,0.708394529056337,1.00061746385361),(1.,
0.708058564166901,1.0006181752469),(1.,0.707430835372077,1.00061950443952),
(1.,0.706796685880364,1.00062084722773)))
REPRESENTATION_ITEM('')
SURFACE()
);
#2565=(
BOUNDED_SURFACE()
B_SPLINE_SURFACE(3,2,((#198825,#198826,#198827),(#198828,#198829,#198830),
(#198831,#198832,#198833),(#198834,#198835,#198836)),.UNSPECIFIED.,.F.,
 .F.,.F.)
B_SPLINE_SURFACE_WITH_KNOTS((4,4),(3,3),(0.,0.000397394465448305),(0.,1.),
 .UNSPECIFIED.)
GEOMETRIC_REPRESENTATION_ITEM()
RATIONAL_B_SPLINE_SURFACE(((1.,0.70549895611075,1.),(1.,0.705821764811781,
1.),(1.,0.706461952521129,1.),(1.,0.707106781186548,1.)))
REPRESENTATION_ITEM('')
SURFACE()
);
#2566=(
BOUNDED_SURFACE()
B_SPLINE_SURFACE(3,2,((#198842,#198843,#198844),(#198845,#198846,#198847),
(#198848,#198849,#198850),(#198851,#198852,#198853)),.UNSPECIFIED.,.F.,
 .F.,.F.)
B_SPLINE_SURFACE_WITH_KNOTS((4,4),(3,3),(0.,0.000397394410828723),(0.,1.),
 .UNSPECIFIED.)
GEOMETRIC_REPRESENTATION_ITEM()
RATIONAL_B_SPLINE_SURFACE(((1.,0.708689770883325,1.),(1.,0.708376440034514,
1.),(1.,0.707750498698386,1.),(1.,0.707106781186546,1.)))
REPRESENTATION_ITEM('')
SURFACE()
);
#2567=(
BOUNDED_SURFACE()
B_SPLINE_SURFACE(3,2,((#198859,#198860,#198861),(#198862,#198863,#198864),
(#198865,#198866,#198867),(#198868,#198869,#198870)),.UNSPECIFIED.,.F.,
 .F.,.F.)
B_SPLINE_SURFACE_WITH_KNOTS((4,4),(3,3),(0.,0.000511815090126178),(0.,1.00105592270211),
 .UNSPECIFIED.)
GEOMETRIC_REPRESENTATION_ITEM()
RATIONAL_B_SPLINE_SURFACE(((1.,0.705266242717508,1.00062243213079),(1.,
0.705584085909156,1.0006217608951),(1.,0.706182089450541,1.00062049800407),
(1.,0.706797508587497,1.000619198334)))
REPRESENTATION_ITEM('')
SURFACE()
);
#2568=(
BOUNDED_SURFACE()
B_SPLINE_SURFACE(3,2,((#198872,#198873,#198874),(#198875,#198876,#198877),
(#198878,#198879,#198880),(#198881,#198882,#198883)),.UNSPECIFIED.,.F.,
 .F.,.F.)
B_SPLINE_SURFACE_WITH_KNOTS((4,4),(3,3),(0.,0.000397394428086619),(0.,1.),
 .UNSPECIFIED.)
GEOMETRIC_REPRESENTATION_ITEM()
RATIONAL_B_SPLINE_SURFACE(((1.,0.707106781186549,1.),(1.,0.706459846759122,
1.),(1.,0.705820510737269,1.),(1.,0.705498956110763,1.)))
REPRESENTATION_ITEM('')
SURFACE()
);
#2569=(
BOUNDED_SURFACE()
B_SPLINE_SURFACE(3,2,((#198889,#198890,#198891),(#198892,#198893,#198894),
(#198895,#198896,#198897),(#198898,#198899,#198900),(#198901,#198902,#198903),
(#198904,#198905,#198906)),.UNSPECIFIED.,.F.,.F.,.F.)
B_SPLINE_SURFACE_WITH_KNOTS((4,2,4),(3,3),(0.,0.000257953807872851,0.000515907615745703),
(0.,1.),.UNSPECIFIED.)
GEOMETRIC_REPRESENTATION_ITEM()
RATIONAL_B_SPLINE_SURFACE(((1.,0.874619707139391,1.),(1.,0.874834349679242,
1.),(1.,0.854686104157454,1.),(1.,0.792476597915482,1.),(1.,0.750887854594861,
1.),(1.,0.70558583803145,1.)))
REPRESENTATION_ITEM('')
SURFACE()
);
#2570=(
BOUNDED_SURFACE()
B_SPLINE_SURFACE(3,2,((#198912,#198913,#198914),(#198915,#198916,#198917),
(#198918,#198919,#198920),(#198921,#198922,#198923)),.UNSPECIFIED.,.F.,
 .F.,.F.)
B_SPLINE_SURFACE_WITH_KNOTS((4,4),(3,3),(0.,0.000511815437699147),(0.,1.00105881331765),
 .UNSPECIFIED.)
GEOMETRIC_REPRESENTATION_ITEM()
RATIONAL_B_SPLINE_SURFACE(((1.,0.706796661945819,1.00062089519822),(1.,
0.707430821224719,1.00061955228564),(1.,0.708058545830186,1.0006182229993),
(1.,0.7083945052522,1.00061751156268)))
REPRESENTATION_ITEM('')
SURFACE()
);
#2571=(
BOUNDED_SURFACE()
B_SPLINE_SURFACE(3,2,((#198925,#198926,#198927),(#198928,#198929,#198930),
(#198931,#198932,#198933),(#198934,#198935,#198936),(#198937,#198938,#198939),
(#198940,#198941,#198942)),.UNSPECIFIED.,.F.,.F.,.F.)
B_SPLINE_SURFACE_WITH_KNOTS((4,2,4),(3,3),(0.,0.00025691531753126,0.00051383063506252),
(0.,1.),.UNSPECIFIED.)
GEOMETRIC_REPRESENTATION_ITEM()
RATIONAL_B_SPLINE_SURFACE(((1.,0.705585838031443,1.),(1.,0.75090243354212,
1.),(1.,0.792329530083374,1.),(1.,0.854288401593351,1.),(1.,0.874998031125783,
1.),(1.,0.874619707139395,1.)))
REPRESENTATION_ITEM('')
SURFACE()
);
#2572=(
BOUNDED_SURFACE()
B_SPLINE_SURFACE(3,2,((#198948,#198949,#198950),(#198951,#198952,#198953),
(#198954,#198955,#198956),(#198957,#198958,#198959),(#198960,#198961,#198962),
(#198963,#198964,#198965)),.UNSPECIFIED.,.F.,.F.,.F.)
B_SPLINE_SURFACE_WITH_KNOTS((4,2,4),(3,3),(-5.77337656848531E-18,0.000256592814262152,
0.00051318562852431),(0.,1.),.UNSPECIFIED.)
GEOMETRIC_REPRESENTATION_ITEM()
RATIONAL_B_SPLINE_SURFACE(((1.,0.708712527163664,1.),(1.,0.753780902613285,
1.),(1.,0.794538995769614,1.),(1.,0.855070770330688,1.),(1.,0.87501842744564,
1.),(1.,0.874619707139388,1.)))
REPRESENTATION_ITEM('')
SURFACE()
);
#2573=(
BOUNDED_SURFACE()
B_SPLINE_SURFACE(3,2,((#198967,#198968,#198969),(#198970,#198971,#198972),
(#198973,#198974,#198975),(#198976,#198977,#198978)),.UNSPECIFIED.,.F.,
 .F.,.F.)
B_SPLINE_SURFACE_WITH_KNOTS((4,4),(3,3),(0.,0.000511815072430395),(0.,1.00105598365917),
 .UNSPECIFIED.)
GEOMETRIC_REPRESENTATION_ITEM()
RATIONAL_B_SPLINE_SURFACE(((1.,0.706797490733591,1.00061923411722),(1.,
0.706182062146506,1.00062053388229),(1.,0.705584062768884,1.00062179683743),
(1.,0.70526622477036,1.00062246810089)))
REPRESENTATION_ITEM('')
SURFACE()
);
#2574=(
BOUNDED_SURFACE()
B_SPLINE_SURFACE(3,2,((#198984,#198985,#198986),(#198987,#198988,#198989),
(#198990,#198991,#198992),(#198993,#198994,#198995),(#198996,#198997,#198998),
(#198999,#199000,#199001)),.UNSPECIFIED.,.F.,.F.,.F.)
B_SPLINE_SURFACE_WITH_KNOTS((4,2,4),(3,3),(-3.13063377305189E-18,0.000257652232350879,
0.00051530446470176),(0.,1.),.UNSPECIFIED.)
GEOMETRIC_REPRESENTATION_ITEM()
RATIONAL_B_SPLINE_SURFACE(((1.,0.874619707139394,1.),(1.,0.874861180430667,
1.),(1.,0.855455725920895,1.),(1.,0.794699358955227,1.),(1.,0.75376897778868,
1.),(1.,0.708712527163649,1.)))
REPRESENTATION_ITEM('')
SURFACE()
);
#2575=(
BOUNDED_SURFACE()
B_SPLINE_SURFACE(3,2,((#199007,#199008,#199009),(#199010,#199011,#199012),
(#199013,#199014,#199015),(#199016,#199017,#199018)),.UNSPECIFIED.,.F.,
 .F.,.F.)
B_SPLINE_SURFACE_WITH_KNOTS((4,4),(3,3),(0.,0.000397394373651914),(0.,1.),
 .UNSPECIFIED.)
GEOMETRIC_REPRESENTATION_ITEM()
RATIONAL_B_SPLINE_SURFACE(((1.,0.707106781186546,1.),(1.,0.707752587915888,
1.),(1.,0.708377654540688,1.),(1.,0.708689770883326,1.)))
REPRESENTATION_ITEM('')
SURFACE()
);
#2576=(
BOUNDED_SURFACE()
B_SPLINE_SURFACE(3,2,((#199020,#199021,#199022),(#199023,#199024,#199025),
(#199026,#199027,#199028),(#199029,#199030,#199031)),.UNSPECIFIED.,.F.,
 .F.,.F.)
B_SPLINE_SURFACE_WITH_KNOTS((4,4),(3,3),(0.,0.000511815456479789),(0.,1.00105873159875),
 .UNSPECIFIED.)
GEOMETRIC_REPRESENTATION_ITEM()
RATIONAL_B_SPLINE_SURFACE(((1.,0.708394529056679,1.00061746385291),(1.,
0.708058564167215,1.0006181752462),(1.,0.707430835372418,1.00061950443882),
(1.,0.706796685880729,1.00062084722703)))
REPRESENTATION_ITEM('')
SURFACE()
);
#2577=(
BOUNDED_SURFACE()
B_SPLINE_SURFACE(3,2,((#199037,#199038,#199039),(#199040,#199041,#199042),
(#199043,#199044,#199045),(#199046,#199047,#199048)),.UNSPECIFIED.,.F.,
 .F.,.F.)
B_SPLINE_SURFACE_WITH_KNOTS((4,4),(3,3),(0.,0.000397394465448298),(0.,1.),
 .UNSPECIFIED.)
GEOMETRIC_REPRESENTATION_ITEM()
RATIONAL_B_SPLINE_SURFACE(((1.,0.705498956110748,1.),(1.,0.705821764811764,
1.),(1.,0.706461952521152,1.),(1.,0.707106781186548,1.)))
REPRESENTATION_ITEM('')
SURFACE()
);
#2578=(
BOUNDED_SURFACE()
B_SPLINE_SURFACE(3,2,((#199054,#199055,#199056),(#199057,#199058,#199059),
(#199060,#199061,#199062),(#199063,#199064,#199065)),.UNSPECIFIED.,.F.,
 .F.,.F.)
B_SPLINE_SURFACE_WITH_KNOTS((4,4),(3,3),(0.,0.000397394410828738),(0.,1.),
 .UNSPECIFIED.)
GEOMETRIC_REPRESENTATION_ITEM()
RATIONAL_B_SPLINE_SURFACE(((1.,0.70868977088332,1.),(1.,0.708376440034514,
1.),(1.,0.707750498698361,1.),(1.,0.70710678118657,1.)))
REPRESENTATION_ITEM('')
SURFACE()
);
#2579=(
BOUNDED_SURFACE()
B_SPLINE_SURFACE(3,2,((#199071,#199072,#199073),(#199074,#199075,#199076),
(#199077,#199078,#199079),(#199080,#199081,#199082)),.UNSPECIFIED.,.F.,
 .F.,.F.)
B_SPLINE_SURFACE_WITH_KNOTS((4,4),(3,3),(0.,0.000511815090126175),(0.,1.00105592270382),
 .UNSPECIFIED.)
GEOMETRIC_REPRESENTATION_ITEM()
RATIONAL_B_SPLINE_SURFACE(((1.,0.705266242717021,1.00062243213179),(1.,
0.705584085908677,1.00062176089611),(1.,0.706182089450028,1.00062049800508),
(1.,0.706797508586997,1.000619198335)))
REPRESENTATION_ITEM('')
SURFACE()
);
#2580=(
BOUNDED_SURFACE()
B_SPLINE_SURFACE(3,2,((#199084,#199085,#199086),(#199087,#199088,#199089),
(#199090,#199091,#199092),(#199093,#199094,#199095)),.UNSPECIFIED.,.F.,
 .F.,.F.)
B_SPLINE_SURFACE_WITH_KNOTS((4,4),(3,3),(0.,0.000397394428086619),(0.,1.),
 .UNSPECIFIED.)
GEOMETRIC_REPRESENTATION_ITEM()
RATIONAL_B_SPLINE_SURFACE(((1.,0.707106781186548,1.),(1.,0.706459846759101,
1.),(1.,0.705820510737285,1.),(1.,0.705498956110761,1.)))
REPRESENTATION_ITEM('')
SURFACE()
);
#2581=(
BOUNDED_SURFACE()
B_SPLINE_SURFACE(3,2,((#199101,#199102,#199103),(#199104,#199105,#199106),
(#199107,#199108,#199109),(#199110,#199111,#199112),(#199113,#199114,#199115),
(#199116,#199117,#199118)),.UNSPECIFIED.,.F.,.F.,.F.)
B_SPLINE_SURFACE_WITH_KNOTS((4,2,4),(3,3),(0.,0.000257953807872853,0.000515907615745706),
(0.,1.),.UNSPECIFIED.)
GEOMETRIC_REPRESENTATION_ITEM()
RATIONAL_B_SPLINE_SURFACE(((1.,0.874619707139386,1.),(1.,0.874834349678556,
1.),(1.,0.854686104158394,1.),(1.,0.792476597914528,1.),(1.,0.750887854595574,
1.),(1.,0.705585838031473,1.)))
REPRESENTATION_ITEM('')
SURFACE()
);
#2582=(
BOUNDED_SURFACE()
B_SPLINE_SURFACE(3,2,((#199124,#199125,#199126),(#199127,#199128,#199129),
(#199130,#199131,#199132),(#199133,#199134,#199135)),.UNSPECIFIED.,.F.,
 .F.,.F.)
B_SPLINE_SURFACE_WITH_KNOTS((4,4),(3,3),(-5.52943107967607E-18,0.000511815437699143),
(0.,1.00105881331528),.UNSPECIFIED.)
GEOMETRIC_REPRESENTATION_ITEM()
RATIONAL_B_SPLINE_SURFACE(((1.,0.706796661946501,1.00062089519683),(1.,
0.707430821225412,1.00061955228425),(1.,0.70805854583087,1.00061822299791),
(1.,0.708394505252892,1.00061751156129)))
REPRESENTATION_ITEM('')
SURFACE()
);
#2583=(
BOUNDED_SURFACE()
B_SPLINE_SURFACE(3,2,((#199137,#199138,#199139),(#199140,#199141,#199142),
(#199143,#199144,#199145),(#199146,#199147,#199148),(#199149,#199150,#199151),
(#199152,#199153,#199154)),.UNSPECIFIED.,.F.,.F.,.F.)
B_SPLINE_SURFACE_WITH_KNOTS((4,2,4),(3,3),(0.,0.000256915317531257,0.000513830635062514),
(0.,1.),.UNSPECIFIED.)
GEOMETRIC_REPRESENTATION_ITEM()
RATIONAL_B_SPLINE_SURFACE(((1.,0.705585838031436,1.),(1.,0.750902433542675,
1.),(1.,0.792329530082598,1.),(1.,0.854288401594112,1.),(1.,0.874998031125178,
1.),(1.,0.874619707139397,1.)))
REPRESENTATION_ITEM('')
SURFACE()
);
#2584=(
BOUNDED_SURFACE()
B_SPLINE_SURFACE(3,2,((#199160,#199161,#199162),(#199163,#199164,#199165),
(#199166,#199167,#199168),(#199169,#199170,#199171),(#199172,#199173,#199174),
(#199175,#199176,#199177)),.UNSPECIFIED.,.F.,.F.,.F.)
B_SPLINE_SURFACE_WITH_KNOTS((4,2,4),(3,3),(0.,0.000256592814262161,0.000513185628524321),
(0.,1.),.UNSPECIFIED.)
GEOMETRIC_REPRESENTATION_ITEM()
RATIONAL_B_SPLINE_SURFACE(((1.,0.70871252716365,1.),(1.,0.753780902613521,
1.),(1.,0.794538995769307,1.),(1.,0.855070770330992,1.),(1.,0.875018427445423,
1.),(1.,0.874619707139387,1.)))
REPRESENTATION_ITEM('')
SURFACE()
);
#2585=(
BOUNDED_SURFACE()
B_SPLINE_SURFACE(3,2,((#199179,#199180,#199181),(#199182,#199183,#199184),
(#199185,#199186,#199187),(#199188,#199189,#199190)),.UNSPECIFIED.,.F.,
 .F.,.F.)
B_SPLINE_SURFACE_WITH_KNOTS((4,4),(3,3),(-2.71050543121376E-20,0.000511815072430412),
(0.,1.00105598365811),.UNSPECIFIED.)
GEOMETRIC_REPRESENTATION_ITEM()
RATIONAL_B_SPLINE_SURFACE(((1.,0.70679749073391,1.0006192341166),(1.,0.706182062146828,
1.00062053388166),(1.,0.705584062769189,1.0006217968368),(1.,0.705266224770668,
1.00062246810027)))
REPRESENTATION_ITEM('')
SURFACE()
);
#2586=(
BOUNDED_SURFACE()
B_SPLINE_SURFACE(3,2,((#199196,#199197,#199198),(#199199,#199200,#199201),
(#199202,#199203,#199204),(#199205,#199206,#199207),(#199208,#199209,#199210),
(#199211,#199212,#199213)),.UNSPECIFIED.,.F.,.F.,.F.)
B_SPLINE_SURFACE_WITH_KNOTS((4,2,4),(3,3),(-1.35525271560688E-20,0.000257652232350877,
0.000515304464701753),(0.,1.),.UNSPECIFIED.)
GEOMETRIC_REPRESENTATION_ITEM()
RATIONAL_B_SPLINE_SURFACE(((1.,0.874619707139393,1.),(1.,0.874861180430549,
1.),(1.,0.855455725921079,1.),(1.,0.794699358955038,1.),(1.,0.753768977788861,
1.),(1.,0.708712527163647,1.)))
REPRESENTATION_ITEM('')
SURFACE()
);
#2587=(
BOUNDED_SURFACE()
B_SPLINE_SURFACE(3,2,((#199219,#199220,#199221),(#199222,#199223,#199224),
(#199225,#199226,#199227),(#199228,#199229,#199230)),.UNSPECIFIED.,.F.,
 .F.,.F.)
B_SPLINE_SURFACE_WITH_KNOTS((4,4),(3,3),(-9.54097911787244E-18,0.000397394373651899),
(0.,1.),.UNSPECIFIED.)
GEOMETRIC_REPRESENTATION_ITEM()
RATIONAL_B_SPLINE_SURFACE(((1.,0.707106781186559,1.),(1.,0.707752587915868,
1.),(1.,0.708377654540717,1.),(1.,0.708689770883331,1.)))
REPRESENTATION_ITEM('')
SURFACE()
);
#2588=(
BOUNDED_SURFACE()
B_SPLINE_SURFACE(3,2,((#199232,#199233,#199234),(#199235,#199236,#199237),
(#199238,#199239,#199240),(#199241,#199242,#199243)),.UNSPECIFIED.,.F.,
 .F.,.F.)
B_SPLINE_SURFACE_WITH_KNOTS((4,4),(3,3),(-6.42389787197661E-18,0.000511815456479784),
(0.,1.00105873159871),.UNSPECIFIED.)
GEOMETRIC_REPRESENTATION_ITEM()
RATIONAL_B_SPLINE_SURFACE(((1.,0.708394529056701,1.00061746385289),(1.,
0.708058564167209,1.00061817524618),(1.,0.707430835372458,1.0006195044388),
(1.,0.706796685880743,1.00062084722701)))
REPRESENTATION_ITEM('')
SURFACE()
);
#2589=(
BOUNDED_SURFACE()
B_SPLINE_SURFACE(3,2,((#199249,#199250,#199251),(#199252,#199253,#199254),
(#199255,#199256,#199257),(#199258,#199259,#199260)),.UNSPECIFIED.,.F.,
 .F.,.F.)
B_SPLINE_SURFACE_WITH_KNOTS((4,4),(3,3),(0.,0.000397394465448303),(0.,1.),
 .UNSPECIFIED.)
GEOMETRIC_REPRESENTATION_ITEM()
RATIONAL_B_SPLINE_SURFACE(((1.,0.705498956110736,1.),(1.,0.705821764811768,
1.),(1.,0.706461952521143,1.),(1.,0.707106781186548,1.)))
REPRESENTATION_ITEM('')
SURFACE()
);
#2590=(
BOUNDED_SURFACE()
B_SPLINE_SURFACE(3,2,((#199266,#199267,#199268),(#199269,#199270,#199271),
(#199272,#199273,#199274),(#199275,#199276,#199277)),.UNSPECIFIED.,.F.,
 .F.,.F.)
B_SPLINE_SURFACE_WITH_KNOTS((4,4),(3,3),(0.,0.00039739441082874),(0.,1.),
 .UNSPECIFIED.)
GEOMETRIC_REPRESENTATION_ITEM()
RATIONAL_B_SPLINE_SURFACE(((1.,0.708689770883341,1.),(1.,0.708376440034484,
1.),(1.,0.707750498698422,1.),(1.,0.707106781186548,1.)))
REPRESENTATION_ITEM('')
SURFACE()
);
#2591=(
BOUNDED_SURFACE()
B_SPLINE_SURFACE(3,2,((#199283,#199284,#199285),(#199286,#199287,#199288),
(#199289,#199290,#199291),(#199292,#199293,#199294)),.UNSPECIFIED.,.F.,
 .F.,.F.)
B_SPLINE_SURFACE_WITH_KNOTS((4,4),(3,3),(0.,0.00051181509012618),(0.,1.0010559227041),
 .UNSPECIFIED.)
GEOMETRIC_REPRESENTATION_ITEM()
RATIONAL_B_SPLINE_SURFACE(((1.,0.705266242716924,1.00062243213196),(1.,
0.705584085908585,1.00062176089628),(1.,0.706182089449929,1.00062049800524),
(1.,0.706797508586937,1.00061919833517)))
REPRESENTATION_ITEM('')
SURFACE()
);
#2592=(
BOUNDED_SURFACE()
B_SPLINE_SURFACE(3,2,((#199296,#199297,#199298),(#199299,#199300,#199301),
(#199302,#199303,#199304),(#199305,#199306,#199307)),.UNSPECIFIED.,.F.,
 .F.,.F.)
B_SPLINE_SURFACE_WITH_KNOTS((4,4),(3,3),(0.,0.00039739442808663),(0.,1.),
 .UNSPECIFIED.)
GEOMETRIC_REPRESENTATION_ITEM()
RATIONAL_B_SPLINE_SURFACE(((1.,0.707106781186535,1.),(1.,0.706459846759098,
1.),(1.,0.705820510737295,1.),(1.,0.705498956110716,1.)))
REPRESENTATION_ITEM('')
SURFACE()
);
#2593=(
BOUNDED_SURFACE()
B_SPLINE_SURFACE(3,2,((#199313,#199314,#199315),(#199316,#199317,#199318),
(#199319,#199320,#199321),(#199322,#199323,#199324),(#199325,#199326,#199327),
(#199328,#199329,#199330)),.UNSPECIFIED.,.F.,.F.,.F.)
B_SPLINE_SURFACE_WITH_KNOTS((4,2,4),(3,3),(0.,0.000257953807872849,0.000515907615745698),
(0.,1.),.UNSPECIFIED.)
GEOMETRIC_REPRESENTATION_ITEM()
RATIONAL_B_SPLINE_SURFACE(((1.,0.874619707139392,1.),(1.,0.874834349679019,
1.),(1.,0.854686104157764,1.),(1.,0.792476597915158,1.),(1.,0.750887854595128,
1.),(1.,0.705585838031423,1.)))
REPRESENTATION_ITEM('')
SURFACE()
);
#2594=(
BOUNDED_SURFACE()
B_SPLINE_SURFACE(3,2,((#199336,#199337,#199338),(#199339,#199340,#199341),
(#199342,#199343,#199344),(#199345,#199346,#199347)),.UNSPECIFIED.,.F.,
 .F.,.F.)
B_SPLINE_SURFACE_WITH_KNOTS((4,4),(3,3),(0.,0.000511815437699143),(0.,1.00105881331394),
 .UNSPECIFIED.)
GEOMETRIC_REPRESENTATION_ITEM()
RATIONAL_B_SPLINE_SURFACE(((1.,0.706796661946904,1.00062089519605),(1.,
0.707430821225788,1.00061955228347),(1.,0.708058545831295,1.00061822299713),
(1.,0.70839450525329,1.00061751156051)))
REPRESENTATION_ITEM('')
SURFACE()
);
#2595=(
BOUNDED_SURFACE()
B_SPLINE_SURFACE(3,2,((#199349,#199350,#199351),(#199352,#199353,#199354),
(#199355,#199356,#199357),(#199358,#199359,#199360),(#199361,#199362,#199363),
(#199364,#199365,#199366)),.UNSPECIFIED.,.F.,.F.,.F.)
B_SPLINE_SURFACE_WITH_KNOTS((4,2,4),(3,3),(2.71050543121376E-20,0.000256915317531268,
0.000513830635062535),(0.,1.),.UNSPECIFIED.)
GEOMETRIC_REPRESENTATION_ITEM()
RATIONAL_B_SPLINE_SURFACE(((1.,0.705585838031462,1.),(1.,0.750902433543319,
1.),(1.,0.792329530081728,1.),(1.,0.854288401595,1.),(1.,0.874998031124529,
1.),(1.,0.874619707139394,1.)))
REPRESENTATION_ITEM('')
SURFACE()
);
#2596=(
BOUNDED_SURFACE()
B_SPLINE_SURFACE(3,2,((#199372,#199373,#199374),(#199375,#199376,#199377),
(#199378,#199379,#199380),(#199381,#199382,#199383),(#199384,#199385,#199386),
(#199387,#199388,#199389)),.UNSPECIFIED.,.F.,.F.,.F.)
B_SPLINE_SURFACE_WITH_KNOTS((4,2,4),(3,3),(-9.32413868337534E-18,0.000256592814262153,
0.000513185628524316),(0.,1.),.UNSPECIFIED.)
GEOMETRIC_REPRESENTATION_ITEM()
RATIONAL_B_SPLINE_SURFACE(((1.,0.708712527163675,1.),(1.,0.753780902613644,
1.),(1.,0.794538995769133,1.),(1.,0.855070770331152,1.),(1.,0.875018427445311,
1.),(1.,0.874619707139391,1.)))
REPRESENTATION_ITEM('')
SURFACE()
);
#2597=(
BOUNDED_SURFACE()
B_SPLINE_SURFACE(3,2,((#199391,#199392,#199393),(#199394,#199395,#199396),
(#199397,#199398,#199399),(#199400,#199401,#199402)),.UNSPECIFIED.,.F.,
 .F.,.F.)
B_SPLINE_SURFACE_WITH_KNOTS((4,4),(3,3),(0.,0.000511815072430403),(0.,1.00105598365889),
 .UNSPECIFIED.)
GEOMETRIC_REPRESENTATION_ITEM()
RATIONAL_B_SPLINE_SURFACE(((1.,0.706797490733682,1.00061923411706),(1.,
0.706182062146602,1.00062053388212),(1.,0.705584062768974,1.00062179683726),
(1.,0.705266224770452,1.00062246810073)))
REPRESENTATION_ITEM('')
SURFACE()
);
#2598=(
BOUNDED_SURFACE()
B_SPLINE_SURFACE(3,2,((#199408,#199409,#199410),(#199411,#199412,#199413),
(#199414,#199415,#199416),(#199417,#199418,#199419),(#199420,#199421,#199422),
(#199423,#199424,#199425)),.UNSPECIFIED.,.F.,.F.,.F.)
B_SPLINE_SURFACE_WITH_KNOTS((4,2,4),(3,3),(0.,0.000257652232350887,0.000515304464701775),
(0.,1.),.UNSPECIFIED.)
GEOMETRIC_REPRESENTATION_ITEM()
RATIONAL_B_SPLINE_SURFACE(((1.,0.874619707139393,1.),(1.,0.874861180430824,
1.),(1.,0.855455725920693,1.),(1.,0.794699358955462,1.),(1.,0.753768977788463,
1.),(1.,0.708712527163685,1.)))
REPRESENTATION_ITEM('')
SURFACE()
);
#2599=(
BOUNDED_SURFACE()
B_SPLINE_SURFACE(3,2,((#199431,#199432,#199433),(#199434,#199435,#199436),
(#199437,#199438,#199439),(#199440,#199441,#199442)),.UNSPECIFIED.,.F.,
 .F.,.F.)
B_SPLINE_SURFACE_WITH_KNOTS((4,4),(3,3),(0.,0.000397394373651918),(0.,1.),
 .UNSPECIFIED.)
GEOMETRIC_REPRESENTATION_ITEM()
RATIONAL_B_SPLINE_SURFACE(((1.,0.707106781186548,1.),(1.,0.707752587915853,
1.),(1.,0.708377654540688,1.),(1.,0.708689770883324,1.)))
REPRESENTATION_ITEM('')
SURFACE()
);
#2600=(
BOUNDED_SURFACE()
B_SPLINE_SURFACE(3,2,((#199444,#199445,#199446),(#199447,#199448,#199449),
(#199450,#199451,#199452),(#199453,#199454,#199455)),.UNSPECIFIED.,.F.,
 .F.,.F.)
B_SPLINE_SURFACE_WITH_KNOTS((4,4),(3,3),(0.,0.00051181545647979),(0.,1.00105873159766),
 .UNSPECIFIED.)
GEOMETRIC_REPRESENTATION_ITEM()
RATIONAL_B_SPLINE_SURFACE(((1.,0.708394529056991,1.00061746385228),(1.,
0.708058564167539,1.00061817524556),(1.,0.707430835372731,1.00061950443818),
(1.,0.70679668588105,1.00062084722639)))
REPRESENTATION_ITEM('')
SURFACE()
);
#2601=(
BOUNDED_SURFACE()
B_SPLINE_SURFACE(3,2,((#199461,#199462,#199463),(#199464,#199465,#199466),
(#199467,#199468,#199469),(#199470,#199471,#199472)),.UNSPECIFIED.,.F.,
 .F.,.F.)
B_SPLINE_SURFACE_WITH_KNOTS((4,4),(3,3),(-6.50521303491303E-18,0.000397394465448297),
(0.,1.),.UNSPECIFIED.)
GEOMETRIC_REPRESENTATION_ITEM()
RATIONAL_B_SPLINE_SURFACE(((1.,0.705498956110752,1.),(1.,0.705821764811808,
1.),(1.,0.706461952521121,1.),(1.,0.707106781186562,1.)))
REPRESENTATION_ITEM('')
SURFACE()
);
#2602=(
BOUNDED_SURFACE()
B_SPLINE_SURFACE(3,2,((#199478,#199479,#199480),(#199481,#199482,#199483),
(#199484,#199485,#199486),(#199487,#199488,#199489)),.UNSPECIFIED.,.F.,
 .F.,.F.)
B_SPLINE_SURFACE_WITH_KNOTS((4,4),(3,3),(0.,0.000397394410828735),(0.,1.),
 .UNSPECIFIED.)
GEOMETRIC_REPRESENTATION_ITEM()
RATIONAL_B_SPLINE_SURFACE(((1.,0.708689770883324,1.),(1.,0.708376440034495,
1.),(1.,0.707750498698409,1.),(1.,0.707106781186548,1.)))
REPRESENTATION_ITEM('')
SURFACE()
);
#2603=(
BOUNDED_SURFACE()
B_SPLINE_SURFACE(3,2,((#199495,#199496,#199497),(#199498,#199499,#199500),
(#199501,#199502,#199503),(#199504,#199505,#199506)),.UNSPECIFIED.,.F.,
 .F.,.F.)
B_SPLINE_SURFACE_WITH_KNOTS((4,4),(3,3),(0.,0.000511815090126181),(0.,1.00105592270387),
 .UNSPECIFIED.)
GEOMETRIC_REPRESENTATION_ITEM()
RATIONAL_B_SPLINE_SURFACE(((1.,0.705266242717002,1.00062243213182),(1.,
0.705584085908638,1.00062176089614),(1.,0.706182089450009,1.00062049800511),
(1.,0.706797508586993,1.00061919833503)))
REPRESENTATION_ITEM('')
SURFACE()
);
#2604=(
BOUNDED_SURFACE()
B_SPLINE_SURFACE(3,2,((#199508,#199509,#199510),(#199511,#199512,#199513),
(#199514,#199515,#199516),(#199517,#199518,#199519)),.UNSPECIFIED.,.F.,
 .F.,.F.)
B_SPLINE_SURFACE_WITH_KNOTS((4,4),(3,3),(-5.09575021068187E-18,0.000397394428086632),
(0.,1.),.UNSPECIFIED.)
GEOMETRIC_REPRESENTATION_ITEM()
RATIONAL_B_SPLINE_SURFACE(((1.,0.707106781186535,1.),(1.,0.70645984675911,
1.),(1.,0.705820510737273,1.),(1.,0.705498956110752,1.)))
REPRESENTATION_ITEM('')
SURFACE()
);
#2605=(
BOUNDED_SURFACE()
B_SPLINE_SURFACE(3,2,((#199525,#199526,#199527),(#199528,#199529,#199530),
(#199531,#199532,#199533),(#199534,#199535,#199536),(#199537,#199538,#199539),
(#199540,#199541,#199542)),.UNSPECIFIED.,.F.,.F.,.F.)
B_SPLINE_SURFACE_WITH_KNOTS((4,2,4),(3,3),(0.,0.000257953807872843,0.000515907615745686),
(0.,1.),.UNSPECIFIED.)
GEOMETRIC_REPRESENTATION_ITEM()
RATIONAL_B_SPLINE_SURFACE(((1.,0.874619707139381,1.),(1.,0.874834349679065,
1.),(1.,0.854686104157677,1.),(1.,0.792476597915275,1.),(1.,0.750887854595022,
1.),(1.,0.705585838031447,1.)))
REPRESENTATION_ITEM('')
SURFACE()
);
#2606=(
BOUNDED_SURFACE()
B_SPLINE_SURFACE(3,2,((#199548,#199549,#199550),(#199551,#199552,#199553),
(#199554,#199555,#199556),(#199557,#199558,#199559)),.UNSPECIFIED.,.F.,
 .F.,.F.)
B_SPLINE_SURFACE_WITH_KNOTS((4,4),(3,3),(-9.64939933512099E-18,0.000511815437699146),
(0.,1.00105881331722),.UNSPECIFIED.)
GEOMETRIC_REPRESENTATION_ITEM()
RATIONAL_B_SPLINE_SURFACE(((1.,0.706796661945945,1.00062089519797),(1.,
0.707430821224828,1.00061955228539),(1.,0.708058545830313,1.00061822299905),
(1.,0.708394505252324,1.00061751156243)))
REPRESENTATION_ITEM('')
SURFACE()
);
#2607=(
BOUNDED_SURFACE()
B_SPLINE_SURFACE(3,2,((#199561,#199562,#199563),(#199564,#199565,#199566),
(#199567,#199568,#199569),(#199570,#199571,#199572),(#199573,#199574,#199575),
(#199576,#199577,#199578)),.UNSPECIFIED.,.F.,.F.,.F.)
B_SPLINE_SURFACE_WITH_KNOTS((4,2,4),(3,3),(0.,0.000256915317531262,0.000513830635062524),
(0.,1.),.UNSPECIFIED.)
GEOMETRIC_REPRESENTATION_ITEM()
RATIONAL_B_SPLINE_SURFACE(((1.,0.705585838031416,1.),(1.,0.750902433542617,
1.),(1.,0.792329530082699,1.),(1.,0.854288401594014,1.),(1.,0.874998031125278,
1.),(1.,0.874619707139387,1.)))
REPRESENTATION_ITEM('')
SURFACE()
);
#2608=(
BOUNDED_SURFACE()
B_SPLINE_SURFACE(3,2,((#199584,#199585,#199586),(#199587,#199588,#199589),
(#199590,#199591,#199592),(#199593,#199594,#199595),(#199596,#199597,#199598),
(#199599,#199600,#199601)),.UNSPECIFIED.,.F.,.F.,.F.)
B_SPLINE_SURFACE_WITH_KNOTS((4,2,4),(3,3),(0.,0.000256592814262154,0.000513185628524309),
(0.,1.),.UNSPECIFIED.)
GEOMETRIC_REPRESENTATION_ITEM()
RATIONAL_B_SPLINE_SURFACE(((1.,0.70871252716366,1.),(1.,0.753780902613466,
1.),(1.,0.794538995769324,1.),(1.,0.855070770330988,1.),(1.,0.875018427445413,
1.),(1.,0.874619707139393,1.)))
REPRESENTATION_ITEM('')
SURFACE()
);
#2609=(
BOUNDED_SURFACE()
B_SPLINE_SURFACE(3,2,((#199603,#199604,#199605),(#199606,#199607,#199608),
(#199609,#199610,#199611),(#199612,#199613,#199614)),.UNSPECIFIED.,.F.,
 .F.,.F.)
B_SPLINE_SURFACE_WITH_KNOTS((4,4),(3,3),(0.,0.000511815072430401),(0.,1.00105598365676),
 .UNSPECIFIED.)
GEOMETRIC_REPRESENTATION_ITEM()
RATIONAL_B_SPLINE_SURFACE(((1.,0.706797490734305,1.00061923411581),(1.,
0.706182062147239,1.00062053388087),(1.,0.705584062769544,1.00062179683601),
(1.,0.705266224771083,1.00062246809947)))
REPRESENTATION_ITEM('')
SURFACE()
);
#2610=(
BOUNDED_SURFACE()
B_SPLINE_SURFACE(3,2,((#199620,#199621,#199622),(#199623,#199624,#199625),
(#199626,#199627,#199628),(#199629,#199630,#199631),(#199632,#199633,#199634),
(#199635,#199636,#199637)),.UNSPECIFIED.,.F.,.F.,.F.)
B_SPLINE_SURFACE_WITH_KNOTS((4,2,4),(3,3),(0.,0.000257652232350877,0.000515304464701754),
(0.,1.),.UNSPECIFIED.)
GEOMETRIC_REPRESENTATION_ITEM()
RATIONAL_B_SPLINE_SURFACE(((1.,0.874619707139381,1.),(1.,0.874861180430772,
1.),(1.,0.855455725920791,1.),(1.,0.794699358955345,1.),(1.,0.753768977788573,
1.),(1.,0.708712527163675,1.)))
REPRESENTATION_ITEM('')
SURFACE()
);
#2611=(
BOUNDED_SURFACE()
B_SPLINE_SURFACE(3,2,((#199643,#199644,#199645),(#199646,#199647,#199648),
(#199649,#199650,#199651),(#199652,#199653,#199654)),.UNSPECIFIED.,.F.,
 .F.,.F.)
B_SPLINE_SURFACE_WITH_KNOTS((4,4),(3,3),(0.,0.000397394373651921),(0.,1.),
 .UNSPECIFIED.)
GEOMETRIC_REPRESENTATION_ITEM()
RATIONAL_B_SPLINE_SURFACE(((1.,0.707106781186548,1.),(1.,0.70775258791592,
1.),(1.,0.708377654540668,1.),(1.,0.70868977088334,1.)))
REPRESENTATION_ITEM('')
SURFACE()
);
#2612=(
BOUNDED_SURFACE()
B_SPLINE_SURFACE(3,2,((#199656,#199657,#199658),(#199659,#199660,#199661),
(#199662,#199663,#199664),(#199665,#199666,#199667)),.UNSPECIFIED.,.F.,
 .F.,.F.)
B_SPLINE_SURFACE_WITH_KNOTS((4,4),(3,3),(0.,0.000511815456479783),(0.,1.00105873159891),
 .UNSPECIFIED.)
GEOMETRIC_REPRESENTATION_ITEM()
RATIONAL_B_SPLINE_SURFACE(((1.,0.708394529056628,1.000617463853),(1.,0.708058564167186,
1.00061817524629),(1.,0.707430835372387,1.00061950443891),(1.,0.706796685880672,
1.00062084722712)))
REPRESENTATION_ITEM('')
SURFACE()
);
#2613=(
BOUNDED_SURFACE()
B_SPLINE_SURFACE(3,2,((#199673,#199674,#199675),(#199676,#199677,#199678),
(#199679,#199680,#199681),(#199682,#199683,#199684)),.UNSPECIFIED.,.F.,
 .F.,.F.)
B_SPLINE_SURFACE_WITH_KNOTS((4,4),(3,3),(0.,0.000397394465448299),(0.,1.),
 .UNSPECIFIED.)
GEOMETRIC_REPRESENTATION_ITEM()
RATIONAL_B_SPLINE_SURFACE(((1.,0.705498956110742,1.),(1.,0.705821764811775,
1.),(1.,0.706461952521124,1.),(1.,0.707106781186548,1.)))
REPRESENTATION_ITEM('')
SURFACE()
);
#2614=(
BOUNDED_SURFACE()
B_SPLINE_SURFACE(3,2,((#199690,#199691,#199692),(#199693,#199694,#199695),
(#199696,#199697,#199698),(#199699,#199700,#199701)),.UNSPECIFIED.,.F.,
 .F.,.F.)
B_SPLINE_SURFACE_WITH_KNOTS((4,4),(3,3),(0.,0.000397394410828729),(0.,1.),
 .UNSPECIFIED.)
GEOMETRIC_REPRESENTATION_ITEM()
RATIONAL_B_SPLINE_SURFACE(((1.,0.708689770883367,1.),(1.,0.708376440034488,
1.),(1.,0.707750498698389,1.),(1.,0.707106781186548,1.)))
REPRESENTATION_ITEM('')
SURFACE()
);
#2615=(
BOUNDED_SURFACE()
B_SPLINE_SURFACE(3,2,((#199707,#199708,#199709),(#199710,#199711,#199712),
(#199713,#199714,#199715),(#199716,#199717,#199718)),.UNSPECIFIED.,.F.,
 .F.,.F.)
B_SPLINE_SURFACE_WITH_KNOTS((4,4),(3,3),(0.,0.000511815090126175),(0.,1.00105592270219),
 .UNSPECIFIED.)
GEOMETRIC_REPRESENTATION_ITEM()
RATIONAL_B_SPLINE_SURFACE(((1.,0.705266242717483,1.00062243213083),(1.,
0.705584085909122,1.00062176089515),(1.,0.706182089450485,1.00062049800412),
(1.,0.706797508587486,1.00061919833404)))
REPRESENTATION_ITEM('')
SURFACE()
);
#2616=(
BOUNDED_SURFACE()
B_SPLINE_SURFACE(3,2,((#199720,#199721,#199722),(#199723,#199724,#199725),
(#199726,#199727,#199728),(#199729,#199730,#199731)),.UNSPECIFIED.,.F.,
 .F.,.F.)
B_SPLINE_SURFACE_WITH_KNOTS((4,4),(3,3),(-5.52943107967607E-18,0.000397394428086625),
(0.,1.),.UNSPECIFIED.)
GEOMETRIC_REPRESENTATION_ITEM()
RATIONAL_B_SPLINE_SURFACE(((1.,0.707106781186548,1.),(1.,0.706459846759112,
1.),(1.,0.705820510737253,1.),(1.,0.705498956110736,1.)))
REPRESENTATION_ITEM('')
SURFACE()
);
#2617=(
BOUNDED_SURFACE()
B_SPLINE_SURFACE(3,2,((#199737,#199738,#199739),(#199740,#199741,#199742),
(#199743,#199744,#199745),(#199746,#199747,#199748),(#199749,#199750,#199751),
(#199752,#199753,#199754)),.UNSPECIFIED.,.F.,.F.,.F.)
B_SPLINE_SURFACE_WITH_KNOTS((4,2,4),(3,3),(0.,0.000257953807872841,0.000515907615745682),
(0.,1.),.UNSPECIFIED.)
GEOMETRIC_REPRESENTATION_ITEM()
RATIONAL_B_SPLINE_SURFACE(((1.,0.874619707139397,1.),(1.,0.874834349678708,
1.),(1.,0.85468610415817,1.),(1.,0.792476597914768,1.),(1.,0.750887854595433,
1.),(1.,0.705585838031436,1.)))
REPRESENTATION_ITEM('')
SURFACE()
);
#2618=(
BOUNDED_SURFACE()
B_SPLINE_SURFACE(3,2,((#199760,#199761,#199762),(#199763,#199764,#199765),
(#199766,#199767,#199768),(#199769,#199770,#199771)),.UNSPECIFIED.,.F.,
 .F.,.F.)
B_SPLINE_SURFACE_WITH_KNOTS((4,4),(3,3),(0.,0.000511815437699146),(0.,1.00105881331768),
 .UNSPECIFIED.)
GEOMETRIC_REPRESENTATION_ITEM()
RATIONAL_B_SPLINE_SURFACE(((1.,0.706796661945808,1.00062089519824),(1.,
0.707430821224685,1.00061955228566),(1.,0.708058545830195,1.00061822299932),
(1.,0.708394505252203,1.0006175115627)))
REPRESENTATION_ITEM('')
SURFACE()
);
#2619=(
BOUNDED_SURFACE()
B_SPLINE_SURFACE(3,2,((#199773,#199774,#199775),(#199776,#199777,#199778),
(#199779,#199780,#199781),(#199782,#199783,#199784),(#199785,#199786,#199787),
(#199788,#199789,#199790)),.UNSPECIFIED.,.F.,.F.,.F.)
B_SPLINE_SURFACE_WITH_KNOTS((4,2,4),(3,3),(-5.77337656848531E-18,0.000256915317531248,
0.000513830635062502),(0.,1.),.UNSPECIFIED.)
GEOMETRIC_REPRESENTATION_ITEM()
RATIONAL_B_SPLINE_SURFACE(((1.,0.705585838031448,1.),(1.,0.750902433542038,
1.),(1.,0.792329530083478,1.),(1.,0.854288401593252,1.),(1.,0.874998031125851,
1.),(1.,0.874619707139389,1.)))
REPRESENTATION_ITEM('')
SURFACE()
);
#2620=(
BOUNDED_SURFACE()
B_SPLINE_SURFACE(3,2,((#199796,#199797,#199798),(#199799,#199800,#199801),
(#199802,#199803,#199804),(#199805,#199806,#199807),(#199808,#199809,#199810),
(#199811,#199812,#199813)),.UNSPECIFIED.,.F.,.F.,.F.)
B_SPLINE_SURFACE_WITH_KNOTS((4,2,4),(3,3),(-8.91756286869327E-18,0.000256592814262157,
0.000513185628524322),(0.,1.),.UNSPECIFIED.)
GEOMETRIC_REPRESENTATION_ITEM()
RATIONAL_B_SPLINE_SURFACE(((1.,0.70871252716367,1.),(1.,0.753780902614205,
1.),(1.,0.794538995768374,1.),(1.,0.855070770331893,1.),(1.,0.875018427444734,
1.),(1.,0.874619707139393,1.)))
REPRESENTATION_ITEM('')
SURFACE()
);
#2621=(
BOUNDED_SURFACE()
B_SPLINE_SURFACE(3,2,((#199815,#199816,#199817),(#199818,#199819,#199820),
(#199821,#199822,#199823),(#199824,#199825,#199826)),.UNSPECIFIED.,.F.,
 .F.,.F.)
B_SPLINE_SURFACE_WITH_KNOTS((4,4),(3,3),(-9.54097911787244E-18,0.000511815072430398),
(0.,1.0010559836562),.UNSPECIFIED.)
GEOMETRIC_REPRESENTATION_ITEM()
RATIONAL_B_SPLINE_SURFACE(((1.,0.70679749073447,1.00061923411548),(1.,0.706182062147385,
1.00062053388054),(1.,0.705584062769784,1.00062179683568),(1.,0.705266224771247,
1.00062246809914)))
REPRESENTATION_ITEM('')
SURFACE()
);
#2622=(
BOUNDED_SURFACE()
B_SPLINE_SURFACE(3,2,((#199832,#199833,#199834),(#199835,#199836,#199837),
(#199838,#199839,#199840),(#199841,#199842,#199843),(#199844,#199845,#199846),
(#199847,#199848,#199849)),.UNSPECIFIED.,.F.,.F.,.F.)
B_SPLINE_SURFACE_WITH_KNOTS((4,2,4),(3,3),(0.,0.000257652232350877,0.000515304464701755),
(0.,1.),.UNSPECIFIED.)
GEOMETRIC_REPRESENTATION_ITEM()
RATIONAL_B_SPLINE_SURFACE(((1.,0.874619707139387,1.),(1.,0.874861180430636,
1.),(1.,0.855455725920972,1.),(1.,0.794699358955189,1.),(1.,0.753768977788693,
1.),(1.,0.70871252716365,1.)))
REPRESENTATION_ITEM('')
SURFACE()
);
#2623=(
BOUNDED_SURFACE()
B_SPLINE_SURFACE(3,2,((#199855,#199856,#199857),(#199858,#199859,#199860),
(#199861,#199862,#199863),(#199864,#199865,#199866)),.UNSPECIFIED.,.F.,
 .F.,.F.)
B_SPLINE_SURFACE_WITH_KNOTS((4,4),(3,3),(-5.52943107967607E-18,0.000397394373651916),
(0.,1.),.UNSPECIFIED.)
GEOMETRIC_REPRESENTATION_ITEM()
RATIONAL_B_SPLINE_SURFACE(((1.,0.707106781186548,1.),(1.,0.707752587915911,
1.),(1.,0.708377654540664,1.),(1.,0.708689770883322,1.)))
REPRESENTATION_ITEM('')
SURFACE()
);
#2624=(
BOUNDED_SURFACE()
B_SPLINE_SURFACE(3,2,((#199868,#199869,#199870),(#199871,#199872,#199873),
(#199874,#199875,#199876),(#199877,#199878,#199879)),.UNSPECIFIED.,.F.,
 .F.,.F.)
B_SPLINE_SURFACE_WITH_KNOTS((4,4),(3,3),(0.,0.000511815456479781),(0.,1.00105873159962),
 .UNSPECIFIED.)
GEOMETRIC_REPRESENTATION_ITEM()
RATIONAL_B_SPLINE_SURFACE(((1.,0.70839452905641,1.00061746385342),(1.,0.708058564166979,
1.00061817524671),(1.,0.707430835372153,1.00061950443933),(1.,0.706796685880476,
1.00062084722754)))
REPRESENTATION_ITEM('')
SURFACE()
);
#2625=(
BOUNDED_SURFACE()
B_SPLINE_SURFACE(3,2,((#199885,#199886,#199887),(#199888,#199889,#199890),
(#199891,#199892,#199893),(#199894,#199895,#199896)),.UNSPECIFIED.,.F.,
 .F.,.F.)
B_SPLINE_SURFACE_WITH_KNOTS((4,4),(3,3),(0.,0.000397394465448313),(0.,1.),
 .UNSPECIFIED.)
GEOMETRIC_REPRESENTATION_ITEM()
RATIONAL_B_SPLINE_SURFACE(((1.,0.705498956110761,1.),(1.,0.705821764811814,
1.),(1.,0.706461952521111,1.),(1.,0.707106781186548,1.)))
REPRESENTATION_ITEM('')
SURFACE()
);
#2626=(
BOUNDED_SURFACE()
B_SPLINE_SURFACE(3,2,((#199902,#199903,#199904),(#199905,#199906,#199907),
(#199908,#199909,#199910),(#199911,#199912,#199913)),.UNSPECIFIED.,.F.,
 .F.,.F.)
B_SPLINE_SURFACE_WITH_KNOTS((4,4),(3,3),(0.,0.000397394410828733),(0.,1.),
 .UNSPECIFIED.)
GEOMETRIC_REPRESENTATION_ITEM()
RATIONAL_B_SPLINE_SURFACE(((1.,0.708689770883358,1.),(1.,0.708376440034475,
1.),(1.,0.707750498698409,1.),(1.,0.707106781186548,1.)))
REPRESENTATION_ITEM('')
SURFACE()
);
#2627=(
BOUNDED_SURFACE()
B_SPLINE_SURFACE(3,2,((#199919,#199920,#199921),(#199922,#199923,#199924),
(#199925,#199926,#199927),(#199928,#199929,#199930)),.UNSPECIFIED.,.F.,
 .F.,.F.)
B_SPLINE_SURFACE_WITH_KNOTS((4,4),(3,3),(0.,0.000511815090126173),(0.,1.00105592270345),
 .UNSPECIFIED.)
GEOMETRIC_REPRESENTATION_ITEM()
RATIONAL_B_SPLINE_SURFACE(((1.,0.705266242717092,1.00062243213157),(1.,
0.7055840859088,1.00062176089589),(1.,0.706182089450108,1.00062049800486),
(1.,0.706797508587117,1.00061919833478)))
REPRESENTATION_ITEM('')
SURFACE()
);
#2628=(
BOUNDED_SURFACE()
B_SPLINE_SURFACE(3,2,((#199932,#199933,#199934),(#199935,#199936,#199937),
(#199938,#199939,#199940),(#199941,#199942,#199943)),.UNSPECIFIED.,.F.,
 .F.,.F.)
B_SPLINE_SURFACE_WITH_KNOTS((4,4),(3,3),(-7.64362531602281E-18,0.000397394428086619),
(0.,1.),.UNSPECIFIED.)
GEOMETRIC_REPRESENTATION_ITEM()
RATIONAL_B_SPLINE_SURFACE(((1.,0.707106781186539,1.),(1.,0.706459846759101,
1.),(1.,0.705820510737287,1.),(1.,0.705498956110748,1.)))
REPRESENTATION_ITEM('')
SURFACE()
);
#2629=(
BOUNDED_SURFACE()
B_SPLINE_SURFACE(3,2,((#199949,#199950,#199951),(#199952,#199953,#199954),
(#199955,#199956,#199957),(#199958,#199959,#199960),(#199961,#199962,#199963),
(#199964,#199965,#199966)),.UNSPECIFIED.,.F.,.F.,.F.)
B_SPLINE_SURFACE_WITH_KNOTS((4,2,4),(3,3),(0.,0.000257953807872845,0.00051590761574569),
(0.,1.),.UNSPECIFIED.)
GEOMETRIC_REPRESENTATION_ITEM()
RATIONAL_B_SPLINE_SURFACE(((1.,0.874619707139383,1.),(1.,0.874834349679653,
1.),(1.,0.854686104156939,1.),(1.,0.792476597916007,1.),(1.,0.750887854594488,
1.),(1.,0.705585838031433,1.)))
REPRESENTATION_ITEM('')
SURFACE()
);
#2630=(
BOUNDED_SURFACE()
B_SPLINE_SURFACE(3,2,((#199972,#199973,#199974),(#199975,#199976,#199977),
(#199978,#199979,#199980),(#199981,#199982,#199983)),.UNSPECIFIED.,.F.,
 .F.,.F.)
B_SPLINE_SURFACE_WITH_KNOTS((4,4),(3,3),(-7.61652026171067E-18,0.000511815437699149),
(0.,1.00105881331741),.UNSPECIFIED.)
GEOMETRIC_REPRESENTATION_ITEM()
RATIONAL_B_SPLINE_SURFACE(((1.,0.706796661945879,1.00062089519808),(1.,
0.707430821224774,1.0006195522855),(1.,0.70805854583029,1.00061822299916),
(1.,0.708394505252249,1.00061751156254)))
REPRESENTATION_ITEM('')
SURFACE()
);
#2631=(
BOUNDED_SURFACE()
B_SPLINE_SURFACE(3,2,((#199985,#199986,#199987),(#199988,#199989,#199990),
(#199991,#199992,#199993),(#199994,#199995,#199996),(#199997,#199998,#199999),
(#200000,#200001,#200002)),.UNSPECIFIED.,.F.,.F.,.F.)
B_SPLINE_SURFACE_WITH_KNOTS((4,2,4),(3,3),(0.,0.000256915317531265,0.000513830635062531),
(0.,1.),.UNSPECIFIED.)
GEOMETRIC_REPRESENTATION_ITEM()
RATIONAL_B_SPLINE_SURFACE(((1.,0.705585838031483,1.),(1.,0.750902433542739,
1.),(1.,0.792329530082514,1.),(1.,0.854288401594209,1.),(1.,0.87499803112514,
1.),(1.,0.874619707139408,1.)))
REPRESENTATION_ITEM('')
SURFACE()
);
#2632=(
BOUNDED_SURFACE()
B_SPLINE_SURFACE(3,2,((#200008,#200009,#200010),(#200011,#200012,#200013),
(#200014,#200015,#200016),(#200017,#200018,#200019),(#200020,#200021,#200022),
(#200023,#200024,#200025)),.UNSPECIFIED.,.F.,.F.,.F.)
B_SPLINE_SURFACE_WITH_KNOTS((4,2,4),(3,3),(0.,0.000256592814262162,0.000513185628524324),
(0.,1.),.UNSPECIFIED.)
GEOMETRIC_REPRESENTATION_ITEM()
RATIONAL_B_SPLINE_SURFACE(((1.,0.708712527163667,1.),(1.,0.753780902613371,
1.),(1.,0.794538995769506,1.),(1.,0.855070770330781,1.),(1.,0.875018427445574,
1.),(1.,0.874619707139391,1.)))
REPRESENTATION_ITEM('')
SURFACE()
);
#2633=(
BOUNDED_SURFACE()
B_SPLINE_SURFACE(3,2,((#200027,#200028,#200029),(#200030,#200031,#200032),
(#200033,#200034,#200035),(#200036,#200037,#200038)),.UNSPECIFIED.,.F.,
 .F.,.F.)
B_SPLINE_SURFACE_WITH_KNOTS((4,4),(3,3),(0.,0.000511815072430398),(0.,1.00105598366041),
 .UNSPECIFIED.)
GEOMETRIC_REPRESENTATION_ITEM()
RATIONAL_B_SPLINE_SURFACE(((1.,0.706797490733237,1.00061923411795),(1.,
0.706182062146155,1.00062053388302),(1.,0.705584062768535,1.00062179683816),
(1.,0.705266224770017,1.00062246810163)))
REPRESENTATION_ITEM('')
SURFACE()
);
#2634=(
BOUNDED_SURFACE()
B_SPLINE_SURFACE(3,2,((#200044,#200045,#200046),(#200047,#200048,#200049),
(#200050,#200051,#200052),(#200053,#200054,#200055),(#200056,#200057,#200058),
(#200059,#200060,#200061)),.UNSPECIFIED.,.F.,.F.,.F.)
B_SPLINE_SURFACE_WITH_KNOTS((4,2,4),(3,3),(0.,0.000257652232350879,0.000515304464701758),
(0.,1.),.UNSPECIFIED.)
GEOMETRIC_REPRESENTATION_ITEM()
RATIONAL_B_SPLINE_SURFACE(((1.,0.874619707139379,1.),(1.,0.87486118043056,
1.),(1.,0.855455725921018,1.),(1.,0.794699358955082,1.),(1.,0.753768977788767,
1.),(1.,0.708712527163641,1.)))
REPRESENTATION_ITEM('')
SURFACE()
);
#2635=(
BOUNDED_SURFACE()
B_SPLINE_SURFACE(3,2,((#200067,#200068,#200069),(#200070,#200071,#200072),
(#200073,#200074,#200075),(#200076,#200077,#200078)),.UNSPECIFIED.,.F.,
 .F.,.F.)
B_SPLINE_SURFACE_WITH_KNOTS((4,4),(3,3),(0.,0.000397394373651927),(0.,1.),
 .UNSPECIFIED.)
GEOMETRIC_REPRESENTATION_ITEM()
RATIONAL_B_SPLINE_SURFACE(((1.,0.707106781186548,1.),(1.,0.707752587915909,
1.),(1.,0.708377654540638,1.),(1.,0.708689770883346,1.)))
REPRESENTATION_ITEM('')
SURFACE()
);
#2636=(
BOUNDED_SURFACE()
B_SPLINE_SURFACE(3,2,((#200080,#200081,#200082),(#200083,#200084,#200085),
(#200086,#200087,#200088),(#200089,#200090,#200091)),.UNSPECIFIED.,.F.,
 .F.,.F.)
B_SPLINE_SURFACE_WITH_KNOTS((4,4),(3,3),(0.,0.000511815456479783),(0.,1.00105873160187),
 .UNSPECIFIED.)
GEOMETRIC_REPRESENTATION_ITEM()
RATIONAL_B_SPLINE_SURFACE(((1.,0.708394529055766,1.00061746385473),(1.,
0.70805856416633,1.00061817524803),(1.,0.707430835371486,1.00061950444065),
(1.,0.706796685879816,1.00062084722886)))
REPRESENTATION_ITEM('')
SURFACE()
);
#2637=(
BOUNDED_SURFACE()
B_SPLINE_SURFACE(3,2,((#200097,#200098,#200099),(#200100,#200101,#200102),
(#200103,#200104,#200105),(#200106,#200107,#200108)),.UNSPECIFIED.,.F.,
 .F.,.F.)
B_SPLINE_SURFACE_WITH_KNOTS((4,4),(3,3),(0.,0.000397394465448308),(0.,1.),
 .UNSPECIFIED.)
GEOMETRIC_REPRESENTATION_ITEM()
RATIONAL_B_SPLINE_SURFACE(((1.,0.705498956110759,1.),(1.,0.705821764811768,
1.),(1.,0.706461952521157,1.),(1.,0.707106781186548,1.)))
REPRESENTATION_ITEM('')
SURFACE()
);
#2638=(
BOUNDED_SURFACE()
B_SPLINE_SURFACE(3,2,((#200114,#200115,#200116),(#200117,#200118,#200119),
(#200120,#200121,#200122),(#200123,#200124,#200125)),.UNSPECIFIED.,.F.,
 .F.,.F.)
B_SPLINE_SURFACE_WITH_KNOTS((4,4),(3,3),(0.,0.000397394410828734),(0.,1.),
 .UNSPECIFIED.)
GEOMETRIC_REPRESENTATION_ITEM()
RATIONAL_B_SPLINE_SURFACE(((1.,0.708689770883336,1.),(1.,0.708376440034494,
1.),(1.,0.70775049869841,1.),(1.,0.707106781186548,1.)))
REPRESENTATION_ITEM('')
SURFACE()
);
#2639=(
BOUNDED_SURFACE()
B_SPLINE_SURFACE(3,2,((#200131,#200132,#200133),(#200134,#200135,#200136),
(#200137,#200138,#200139),(#200140,#200141,#200142)),.UNSPECIFIED.,.F.,
 .F.,.F.)
B_SPLINE_SURFACE_WITH_KNOTS((4,4),(3,3),(0.,0.000511815090126178),(0.,1.00105592270253),
 .UNSPECIFIED.)
GEOMETRIC_REPRESENTATION_ITEM()
RATIONAL_B_SPLINE_SURFACE(((1.,0.705266242717381,1.00062243213103),(1.,
0.705584085909037,1.00062176089535),(1.,0.706182089450398,1.00062049800432),
(1.,0.706797508587385,1.00061919833424)))
REPRESENTATION_ITEM('')
SURFACE()
);
#2640=(
BOUNDED_SURFACE()
B_SPLINE_SURFACE(3,2,((#200144,#200145,#200146),(#200147,#200148,#200149),
(#200150,#200151,#200152),(#200153,#200154,#200155)),.UNSPECIFIED.,.F.,
 .F.,.F.)
B_SPLINE_SURFACE_WITH_KNOTS((4,4),(3,3),(-1.52601455777335E-17,0.000397394428086621),
(0.,1.),.UNSPECIFIED.)
GEOMETRIC_REPRESENTATION_ITEM()
RATIONAL_B_SPLINE_SURFACE(((1.,0.707106781186548,1.),(1.,0.706459846759085,
1.),(1.,0.705820510737268,1.),(1.,0.70549895611075,1.)))
REPRESENTATION_ITEM('')
SURFACE()
);
#2641=(
BOUNDED_SURFACE()
B_SPLINE_SURFACE(3,2,((#200161,#200162,#200163),(#200164,#200165,#200166),
(#200167,#200168,#200169),(#200170,#200171,#200172),(#200173,#200174,#200175),
(#200176,#200177,#200178)),.UNSPECIFIED.,.F.,.F.,.F.)
B_SPLINE_SURFACE_WITH_KNOTS((4,2,4),(3,3),(0.,0.000257953807872852,0.000515907615745704),
(0.,1.),.UNSPECIFIED.)
GEOMETRIC_REPRESENTATION_ITEM()
RATIONAL_B_SPLINE_SURFACE(((1.,0.874619707139392,1.),(1.,0.874834349679401,
1.),(1.,0.854686104157248,1.),(1.,0.79247659791567,1.),(1.,0.75088785459474,
1.),(1.,0.705585838031443,1.)))
REPRESENTATION_ITEM('')
SURFACE()
);
#2642=(
BOUNDED_SURFACE()
B_SPLINE_SURFACE(3,2,((#200184,#200185,#200186),(#200187,#200188,#200189),
(#200190,#200191,#200192),(#200193,#200194,#200195)),.UNSPECIFIED.,.F.,
 .F.,.F.)
B_SPLINE_SURFACE_WITH_KNOTS((4,4),(3,3),(0.,0.000511815437699151),(0.,1.00105881331662),
 .UNSPECIFIED.)
GEOMETRIC_REPRESENTATION_ITEM()
RATIONAL_B_SPLINE_SURFACE(((1.,0.706796661946136,1.00062089519762),(1.,
0.707430821224989,1.00061955228504),(1.,0.708058545830515,1.0006182229987),
(1.,0.708394505252514,1.00061751156208)))
REPRESENTATION_ITEM('')
SURFACE()
);
#2643=(
BOUNDED_SURFACE()
B_SPLINE_SURFACE(3,2,((#200197,#200198,#200199),(#200200,#200201,#200202),
(#200203,#200204,#200205),(#200206,#200207,#200208),(#200209,#200210,#200211),
(#200212,#200213,#200214)),.UNSPECIFIED.,.F.,.F.,.F.)
B_SPLINE_SURFACE_WITH_KNOTS((4,2,4),(3,3),(0.,0.000256915317531256,0.000513830635062512),
(0.,1.),.UNSPECIFIED.)
GEOMETRIC_REPRESENTATION_ITEM()
RATIONAL_B_SPLINE_SURFACE(((1.,0.705585838031448,1.),(1.,0.750902433542508,
1.),(1.,0.792329530082831,1.),(1.,0.854288401593858,1.),(1.,0.874998031125374,
1.),(1.,0.874619707139394,1.)))
REPRESENTATION_ITEM('')
SURFACE()
);
#2644=(
BOUNDED_SURFACE()
B_SPLINE_SURFACE(3,2,((#200220,#200221,#200222),(#200223,#200224,#200225),
(#200226,#200227,#200228),(#200229,#200230,#200231),(#200232,#200233,#200234),
(#200235,#200236,#200237)),.UNSPECIFIED.,.F.,.F.,.F.)
B_SPLINE_SURFACE_WITH_KNOTS((4,2,4),(3,3),(0.,0.000256592814262157,0.000513185628524313),
(0.,1.),.UNSPECIFIED.)
GEOMETRIC_REPRESENTATION_ITEM()
RATIONAL_B_SPLINE_SURFACE(((1.,0.708712527163664,1.),(1.,0.753780902613601,
1.),(1.,0.794538995769178,1.),(1.,0.855070770331139,1.),(1.,0.8750184274453,
1.),(1.,0.87461970713939,1.)))
REPRESENTATION_ITEM('')
SURFACE()
);
#2645=(
BOUNDED_SURFACE()
B_SPLINE_SURFACE(3,2,((#200239,#200240,#200241),(#200242,#200243,#200244),
(#200245,#200246,#200247),(#200248,#200249,#200250)),.UNSPECIFIED.,.F.,
 .F.,.F.)
B_SPLINE_SURFACE_WITH_KNOTS((4,4),(3,3),(-7.61652026171067E-18,0.000511815072430393),
(0.,1.00105598365944),.UNSPECIFIED.)
GEOMETRIC_REPRESENTATION_ITEM()
RATIONAL_B_SPLINE_SURFACE(((1.,0.70679749073352,1.00061923411738),(1.,0.706182062146414,
1.00062053388245),(1.,0.705584062768852,1.00062179683759),(1.,0.705266224770258,
1.00062246810105)))
REPRESENTATION_ITEM('')
SURFACE()
);
#2646=(
BOUNDED_SURFACE()
B_SPLINE_SURFACE(3,2,((#200256,#200257,#200258),(#200259,#200260,#200261),
(#200262,#200263,#200264),(#200265,#200266,#200267),(#200268,#200269,#200270),
(#200271,#200272,#200273)),.UNSPECIFIED.,.F.,.F.,.F.)
B_SPLINE_SURFACE_WITH_KNOTS((4,2,4),(3,3),(0.,0.000257652232350884,0.000515304464701767),
(0.,1.),.UNSPECIFIED.)
GEOMETRIC_REPRESENTATION_ITEM()
RATIONAL_B_SPLINE_SURFACE(((1.,0.874619707139383,1.),(1.,0.874861180430228,
1.),(1.,0.855455725921542,1.),(1.,0.794699358954615,1.),(1.,0.75376897778914,
1.),(1.,0.708712527163655,1.)))
REPRESENTATION_ITEM('')
SURFACE()
);
#2647=(
BOUNDED_SURFACE()
B_SPLINE_SURFACE(3,2,((#200279,#200280,#200281),(#200282,#200283,#200284),
(#200285,#200286,#200287),(#200288,#200289,#200290)),.UNSPECIFIED.,.F.,
 .F.,.F.)
B_SPLINE_SURFACE_WITH_KNOTS((4,4),(3,3),(0.,0.000397394373651933),(0.,1.),
 .UNSPECIFIED.)
GEOMETRIC_REPRESENTATION_ITEM()
RATIONAL_B_SPLINE_SURFACE(((1.,0.707106781186555,1.),(1.,0.70775258791589,
1.),(1.,0.708377654540668,1.),(1.,0.708689770883335,1.)))
REPRESENTATION_ITEM('')
SURFACE()
);
#2648=(
BOUNDED_SURFACE()
B_SPLINE_SURFACE(3,2,((#200292,#200293,#200294),(#200295,#200296,#200297),
(#200298,#200299,#200300),(#200301,#200302,#200303)),.UNSPECIFIED.,.F.,
 .F.,.F.)
B_SPLINE_SURFACE_WITH_KNOTS((4,4),(3,3),(0.,0.000511815456479785),(0.,1.00105873159945),
 .UNSPECIFIED.)
GEOMETRIC_REPRESENTATION_ITEM()
RATIONAL_B_SPLINE_SURFACE(((1.,0.70839452905647,1.00061746385332),(1.,0.708058564167016,
1.00061817524661),(1.,0.707430835372208,1.00061950443923),(1.,0.706796685880517,
1.00062084722744)))
REPRESENTATION_ITEM('')
SURFACE()
);
#2649=(
BOUNDED_SURFACE()
B_SPLINE_SURFACE(3,2,((#200309,#200310,#200311),(#200312,#200313,#200314),
(#200315,#200316,#200317),(#200318,#200319,#200320)),.UNSPECIFIED.,.F.,
 .F.,.F.)
B_SPLINE_SURFACE_WITH_KNOTS((4,4),(3,3),(0.,0.000397394465448311),(0.,1.),
 .UNSPECIFIED.)
GEOMETRIC_REPRESENTATION_ITEM()
RATIONAL_B_SPLINE_SURFACE(((1.,0.705498956110775,1.),(1.,0.705821764811747,
1.),(1.,0.706461952521171,1.),(1.,0.707106781186548,1.)))
REPRESENTATION_ITEM('')
SURFACE()
);
#2650=(
BOUNDED_SURFACE()
B_SPLINE_SURFACE(3,2,((#200326,#200327,#200328),(#200329,#200330,#200331),
(#200332,#200333,#200334),(#200335,#200336,#200337)),.UNSPECIFIED.,.F.,
 .F.,.F.)
B_SPLINE_SURFACE_WITH_KNOTS((4,4),(3,3),(0.,0.000397394410828724),(0.,1.),
 .UNSPECIFIED.)
GEOMETRIC_REPRESENTATION_ITEM()
RATIONAL_B_SPLINE_SURFACE(((1.,0.708689770883335,1.),(1.,0.708376440034495,
1.),(1.,0.707750498698407,1.),(1.,0.707106781186548,1.)))
REPRESENTATION_ITEM('')
SURFACE()
);
#2651=(
BOUNDED_SURFACE()
B_SPLINE_SURFACE(3,2,((#200343,#200344,#200345),(#200346,#200347,#200348),
(#200349,#200350,#200351),(#200352,#200353,#200354)),.UNSPECIFIED.,.F.,
 .F.,.F.)
B_SPLINE_SURFACE_WITH_KNOTS((4,4),(3,3),(-6.42389787197661E-18,0.000511815090126184),
(0.,1.00105592270257),.UNSPECIFIED.)
GEOMETRIC_REPRESENTATION_ITEM()
RATIONAL_B_SPLINE_SURFACE(((1.,0.705266242717368,1.00062243213106),(1.,
0.705584085909023,1.00062176089537),(1.,0.706182089450383,1.00062049800434),
(1.,0.706797508587373,1.00061919833427)))
REPRESENTATION_ITEM('')
SURFACE()
);
#2652=(
BOUNDED_SURFACE()
B_SPLINE_SURFACE(3,2,((#200356,#200357,#200358),(#200359,#200360,#200361),
(#200362,#200363,#200364),(#200365,#200366,#200367)),.UNSPECIFIED.,.F.,
 .F.,.F.)
B_SPLINE_SURFACE_WITH_KNOTS((4,4),(3,3),(0.,0.000397394428086622),(0.,1.),
 .UNSPECIFIED.)
GEOMETRIC_REPRESENTATION_ITEM()
RATIONAL_B_SPLINE_SURFACE(((1.,0.707106781186548,1.),(1.,0.70645984675908,
1.),(1.,0.705820510737275,1.),(1.,0.705498956110738,1.)))
REPRESENTATION_ITEM('')
SURFACE()
);
#2653=(
BOUNDED_SURFACE()
B_SPLINE_SURFACE(3,2,((#200373,#200374,#200375),(#200376,#200377,#200378),
(#200379,#200380,#200381),(#200382,#200383,#200384),(#200385,#200386,#200387),
(#200388,#200389,#200390)),.UNSPECIFIED.,.F.,.F.,.F.)
B_SPLINE_SURFACE_WITH_KNOTS((4,2,4),(3,3),(0.,0.000257953807872845,0.000515907615745689),
(0.,1.),.UNSPECIFIED.)
GEOMETRIC_REPRESENTATION_ITEM()
RATIONAL_B_SPLINE_SURFACE(((1.,0.874619707139392,1.),(1.,0.874834349679044,
1.),(1.,0.854686104157737,1.),(1.,0.79247659791519,1.),(1.,0.750887854595087,
1.),(1.,0.705585838031451,1.)))
REPRESENTATION_ITEM('')
SURFACE()
);
#2654=(
BOUNDED_SURFACE()
B_SPLINE_SURFACE(3,2,((#200396,#200397,#200398),(#200399,#200400,#200401),
(#200402,#200403,#200404),(#200405,#200406,#200407)),.UNSPECIFIED.,.F.,
 .F.,.F.)
B_SPLINE_SURFACE_WITH_KNOTS((4,4),(3,3),(-7.56231015308639E-18,0.00051181543769915),
(0.,1.00105881331788),.UNSPECIFIED.)
GEOMETRIC_REPRESENTATION_ITEM()
RATIONAL_B_SPLINE_SURFACE(((1.,0.706796661945751,1.00062089519836),(1.,
0.707430821224625,1.00061955228578),(1.,0.708058545830148,1.00061822299943),
(1.,0.708394505252144,1.00061751156281)))
REPRESENTATION_ITEM('')
SURFACE()
);
#2655=(
BOUNDED_SURFACE()
B_SPLINE_SURFACE(3,2,((#200409,#200410,#200411),(#200412,#200413,#200414),
(#200415,#200416,#200417),(#200418,#200419,#200420),(#200421,#200422,#200423),
(#200424,#200425,#200426)),.UNSPECIFIED.,.F.,.F.,.F.)
B_SPLINE_SURFACE_WITH_KNOTS((4,2,4),(3,3),(0.,0.000256915317531263,0.000513830635062527),
(0.,1.),.UNSPECIFIED.)
GEOMETRIC_REPRESENTATION_ITEM()
RATIONAL_B_SPLINE_SURFACE(((1.,0.705585838031485,1.),(1.,0.750902433542256,
1.),(1.,0.792329530083194,1.),(1.,0.854288401593554,1.),(1.,0.874998031125639,
1.),(1.,0.874619707139405,1.)))
REPRESENTATION_ITEM('')
SURFACE()
);
#2656=(
BOUNDED_SURFACE()
B_SPLINE_SURFACE(3,2,((#200432,#200433,#200434),(#200435,#200436,#200437),
(#200438,#200439,#200440),(#200441,#200442,#200443),(#200444,#200445,#200446),
(#200447,#200448,#200449)),.UNSPECIFIED.,.F.,.F.,.F.)
B_SPLINE_SURFACE_WITH_KNOTS((4,2,4),(3,3),(-6.93889390390723E-18,0.000256592814262155,
0.000513185628524316),(0.,1.),.UNSPECIFIED.)
GEOMETRIC_REPRESENTATION_ITEM()
RATIONAL_B_SPLINE_SURFACE(((1.,0.708712527163686,1.),(1.,0.75378090261287,
1.),(1.,0.794538995770134,1.),(1.,0.855070770330187,1.),(1.,0.875018427446025,
1.),(1.,0.874619707139389,1.)))
REPRESENTATION_ITEM('')
SURFACE()
);
#2657=(
BOUNDED_SURFACE()
B_SPLINE_SURFACE(3,2,((#200451,#200452,#200453),(#200454,#200455,#200456),
(#200457,#200458,#200459),(#200460,#200461,#200462)),.UNSPECIFIED.,.F.,
 .F.,.F.)
B_SPLINE_SURFACE_WITH_KNOTS((4,4),(3,3),(-7.56231015308639E-18,0.000511815072430404),
(0.,1.00105598365537),.UNSPECIFIED.)
GEOMETRIC_REPRESENTATION_ITEM()
RATIONAL_B_SPLINE_SURFACE(((1.,0.706797490734704,1.000619234115),(1.,0.706182062147624,
1.00062053388006),(1.,0.70558406277,1.00062179683519),(1.,0.70526622477148,
1.00062246809866)))
REPRESENTATION_ITEM('')
SURFACE()
);
#2658=(
BOUNDED_SURFACE()
B_SPLINE_SURFACE(3,2,((#200468,#200469,#200470),(#200471,#200472,#200473),
(#200474,#200475,#200476),(#200477,#200478,#200479),(#200480,#200481,#200482),
(#200483,#200484,#200485)),.UNSPECIFIED.,.F.,.F.,.F.)
B_SPLINE_SURFACE_WITH_KNOTS((4,2,4),(3,3),(0.,0.000257652232350885,0.000515304464701771),
(0.,1.),.UNSPECIFIED.)
GEOMETRIC_REPRESENTATION_ITEM()
RATIONAL_B_SPLINE_SURFACE(((1.,0.874619707139378,1.),(1.,0.874861180430567,
1.),(1.,0.855455725921006,1.),(1.,0.794699358955097,1.),(1.,0.753768977788738,
1.),(1.,0.708712527163638,1.)))
REPRESENTATION_ITEM('')
SURFACE()
);
#2659=(
BOUNDED_SURFACE()
B_SPLINE_SURFACE(3,2,((#200491,#200492,#200493),(#200494,#200495,#200496),
(#200497,#200498,#200499),(#200500,#200501,#200502)),.UNSPECIFIED.,.F.,
 .F.,.F.)
B_SPLINE_SURFACE_WITH_KNOTS((4,4),(3,3),(-7.58941520739853E-18,0.0003973943736519),
(0.,1.),.UNSPECIFIED.)
GEOMETRIC_REPRESENTATION_ITEM()
RATIONAL_B_SPLINE_SURFACE(((1.,0.707106781186536,1.),(1.,0.707752587915898,
1.),(1.,0.708377654540667,1.),(1.,0.708689770883327,1.)))
REPRESENTATION_ITEM('')
SURFACE()
);
#2660=(
BOUNDED_SURFACE()
B_SPLINE_SURFACE(3,2,((#200504,#200505,#200506),(#200507,#200508,#200509),
(#200510,#200511,#200512),(#200513,#200514,#200515)),.UNSPECIFIED.,.F.,
 .F.,.F.)
B_SPLINE_SURFACE_WITH_KNOTS((4,4),(3,3),(0.,0.000511815456479782),(0.,1.00105873159924),
 .UNSPECIFIED.)
GEOMETRIC_REPRESENTATION_ITEM()
RATIONAL_B_SPLINE_SURFACE(((1.,0.708394529056535,1.0006174638532),(1.,0.708058564167083,
1.00061817524649),(1.,0.707430835372263,1.00061950443911),(1.,0.706796685880587,
1.00062084722732)))
REPRESENTATION_ITEM('')
SURFACE()
);
#2661=(
BOUNDED_SURFACE()
B_SPLINE_SURFACE(3,2,((#200521,#200522,#200523),(#200524,#200525,#200526),
(#200527,#200528,#200529),(#200530,#200531,#200532)),.UNSPECIFIED.,.F.,
 .F.,.F.)
B_SPLINE_SURFACE_WITH_KNOTS((4,4),(3,3),(0.,0.000397394465448297),(0.,1.),
 .UNSPECIFIED.)
GEOMETRIC_REPRESENTATION_ITEM()
RATIONAL_B_SPLINE_SURFACE(((1.,0.705498956110763,1.),(1.,0.705821764811784,
1.),(1.,0.706461952521129,1.),(1.,0.707106781186553,1.)))
REPRESENTATION_ITEM('')
SURFACE()
);
#2662=(
BOUNDED_SURFACE()
B_SPLINE_SURFACE(3,2,((#200538,#200539,#200540),(#200541,#200542,#200543),
(#200544,#200545,#200546),(#200547,#200548,#200549)),.UNSPECIFIED.,.F.,
 .F.,.F.)
B_SPLINE_SURFACE_WITH_KNOTS((4,4),(3,3),(0.,0.000397394410828749),(0.,1.),
 .UNSPECIFIED.)
GEOMETRIC_REPRESENTATION_ITEM()
RATIONAL_B_SPLINE_SURFACE(((1.,0.708689770883354,1.),(1.,0.708376440034453,
1.),(1.,0.70775049869843,1.),(1.,0.707106781186548,1.)))
REPRESENTATION_ITEM('')
SURFACE()
);
#2663=(
BOUNDED_SURFACE()
B_SPLINE_SURFACE(3,2,((#200555,#200556,#200557),(#200558,#200559,#200560),
(#200561,#200562,#200563),(#200564,#200565,#200566)),.UNSPECIFIED.,.F.,
 .F.,.F.)
B_SPLINE_SURFACE_WITH_KNOTS((4,4),(3,3),(0.,0.000511815090126162),(0.,1.00105592270184),
 .UNSPECIFIED.)
GEOMETRIC_REPRESENTATION_ITEM()
RATIONAL_B_SPLINE_SURFACE(((1.,0.705266242717591,1.00062243213062),(1.,
0.705584085909254,1.00062176089494),(1.,0.706182089450601,1.00062049800391),
(1.,0.706797508587589,1.00061919833383)))
REPRESENTATION_ITEM('')
SURFACE()
);
#2664=(
BOUNDED_SURFACE()
B_SPLINE_SURFACE(3,2,((#200568,#200569,#200570),(#200571,#200572,#200573),
(#200574,#200575,#200576),(#200577,#200578,#200579)),.UNSPECIFIED.,.F.,
 .F.,.F.)
B_SPLINE_SURFACE_WITH_KNOTS((4,4),(3,3),(0.,0.000397394428086619),(0.,1.),
 .UNSPECIFIED.)
GEOMETRIC_REPRESENTATION_ITEM()
RATIONAL_B_SPLINE_SURFACE(((1.,0.707106781186543,1.),(1.,0.706459846759101,
1.),(1.,0.705820510737265,1.),(1.,0.705498956110755,1.)))
REPRESENTATION_ITEM('')
SURFACE()
);
#2665=(
BOUNDED_SURFACE()
B_SPLINE_SURFACE(3,2,((#200585,#200586,#200587),(#200588,#200589,#200590),
(#200591,#200592,#200593),(#200594,#200595,#200596),(#200597,#200598,#200599),
(#200600,#200601,#200602)),.UNSPECIFIED.,.F.,.F.,.F.)
B_SPLINE_SURFACE_WITH_KNOTS((4,2,4),(3,3),(0.,0.000257953807872845,0.00051590761574569),
(0.,1.),.UNSPECIFIED.)
GEOMETRIC_REPRESENTATION_ITEM()
RATIONAL_B_SPLINE_SURFACE(((1.,0.874619707139385,1.),(1.,0.874834349679072,
1.),(1.,0.854686104157708,1.),(1.,0.792476597915247,1.),(1.,0.750887854595038,
1.),(1.,0.705585838031441,1.)))
REPRESENTATION_ITEM('')
SURFACE()
);
#2666=(
BOUNDED_SURFACE()
B_SPLINE_SURFACE(3,2,((#200608,#200609,#200610),(#200611,#200612,#200613),
(#200614,#200615,#200616),(#200617,#200618,#200619)),.UNSPECIFIED.,.F.,
 .F.,.F.)
B_SPLINE_SURFACE_WITH_KNOTS((4,4),(3,3),(0.,0.000511815437699156),(0.,1.00105881331423),
 .UNSPECIFIED.)
GEOMETRIC_REPRESENTATION_ITEM()
RATIONAL_B_SPLINE_SURFACE(((1.,0.706796661946819,1.00062089519622),(1.,
0.707430821225705,1.00061955228364),(1.,0.708058545831191,1.0006182229973),
(1.,0.708394505253199,1.00061751156068)))
REPRESENTATION_ITEM('')
SURFACE()
);
#2667=(
BOUNDED_SURFACE()
B_SPLINE_SURFACE(3,2,((#200621,#200622,#200623),(#200624,#200625,#200626),
(#200627,#200628,#200629),(#200630,#200631,#200632),(#200633,#200634,#200635),
(#200636,#200637,#200638)),.UNSPECIFIED.,.F.,.F.,.F.)
B_SPLINE_SURFACE_WITH_KNOTS((4,2,4),(3,3),(-2.71050543121376E-20,0.000256915317531268,
0.000513830635062536),(0.,1.),.UNSPECIFIED.)
GEOMETRIC_REPRESENTATION_ITEM()
RATIONAL_B_SPLINE_SURFACE(((1.,0.705585838031435,1.),(1.,0.750902433542923,
1.),(1.,0.792329530082311,1.),(1.,0.85428840159443,1.),(1.,0.874998031124965,
1.),(1.,0.874619707139413,1.)))
REPRESENTATION_ITEM('')
SURFACE()
);
#2668=(
BOUNDED_SURFACE()
B_SPLINE_SURFACE(3,2,((#200644,#200645,#200646),(#200647,#200648,#200649),
(#200650,#200651,#200652),(#200653,#200654,#200655),(#200656,#200657,#200658),
(#200659,#200660,#200661)),.UNSPECIFIED.,.F.,.F.,.F.)
B_SPLINE_SURFACE_WITH_KNOTS((4,2,4),(3,3),(0.,0.00025659281426216,0.000513185628524319),
(0.,1.),.UNSPECIFIED.)
GEOMETRIC_REPRESENTATION_ITEM()
RATIONAL_B_SPLINE_SURFACE(((1.,0.708712527163666,1.),(1.,0.753780902613624,
1.),(1.,0.794538995769114,1.),(1.,0.8550707703312,1.),(1.,0.875018427445238,
1.),(1.,0.874619707139389,1.)))
REPRESENTATION_ITEM('')
SURFACE()
);
#2669=(
BOUNDED_SURFACE()
B_SPLINE_SURFACE(3,2,((#200663,#200664,#200665),(#200666,#200667,#200668),
(#200669,#200670,#200671),(#200672,#200673,#200674)),.UNSPECIFIED.,.F.,
 .F.,.F.)
B_SPLINE_SURFACE_WITH_KNOTS((4,4),(3,3),(0.,0.000511815072430393),(0.,1.001055983657),
 .UNSPECIFIED.)
GEOMETRIC_REPRESENTATION_ITEM()
RATIONAL_B_SPLINE_SURFACE(((1.,0.706797490734239,1.00061923411595),(1.,
0.706182062147121,1.00062053388101),(1.,0.705584062769543,1.00062179683615),
(1.,0.705266224770998,1.00062246809961)))
REPRESENTATION_ITEM('')
SURFACE()
);
#2670=(
BOUNDED_SURFACE()
B_SPLINE_SURFACE(3,2,((#200680,#200681,#200682),(#200683,#200684,#200685),
(#200686,#200687,#200688),(#200689,#200690,#200691),(#200692,#200693,#200694),
(#200695,#200696,#200697)),.UNSPECIFIED.,.F.,.F.,.F.)
B_SPLINE_SURFACE_WITH_KNOTS((4,2,4),(3,3),(0.,0.000257652232350883,0.000515304464701766),
(0.,1.),.UNSPECIFIED.)
GEOMETRIC_REPRESENTATION_ITEM()
RATIONAL_B_SPLINE_SURFACE(((1.,0.874619707139393,1.),(1.,0.87486118043087,
1.),(1.,0.85545572592062,1.),(1.,0.794699358955489,1.),(1.,0.753768977788488,
1.),(1.,0.708712527163643,1.)))
REPRESENTATION_ITEM('')
SURFACE()
);
#2671=(
BOUNDED_SURFACE()
B_SPLINE_SURFACE(3,2,((#200703,#200704,#200705),(#200706,#200707,#200708),
(#200709,#200710,#200711),(#200712,#200713,#200714)),.UNSPECIFIED.,.F.,
 .F.,.F.)
B_SPLINE_SURFACE_WITH_KNOTS((4,4),(3,3),(0.,0.00039739437365191),(0.,1.),
 .UNSPECIFIED.)
GEOMETRIC_REPRESENTATION_ITEM()
RATIONAL_B_SPLINE_SURFACE(((1.,0.707106781186552,1.),(1.,0.707752587915889,
1.),(1.,0.708377654540681,1.),(1.,0.708689770883327,1.)))
REPRESENTATION_ITEM('')
SURFACE()
);
#2672=(
BOUNDED_SURFACE()
B_SPLINE_SURFACE(3,2,((#200716,#200717,#200718),(#200719,#200720,#200721),
(#200722,#200723,#200724),(#200725,#200726,#200727)),.UNSPECIFIED.,.F.,
 .F.,.F.)
B_SPLINE_SURFACE_WITH_KNOTS((4,4),(3,3),(-6.42389787197661E-18,0.000511815456479792),
(0.,1.00105873159888),.UNSPECIFIED.)
GEOMETRIC_REPRESENTATION_ITEM()
RATIONAL_B_SPLINE_SURFACE(((1.,0.708394529056643,1.00061746385299),(1.,
0.708058564167205,1.00061817524628),(1.,0.707430835372362,1.0006195044389),
(1.,0.706796685880692,1.00062084722711)))
REPRESENTATION_ITEM('')
SURFACE()
);
#2673=(
BOUNDED_SURFACE()
B_SPLINE_SURFACE(3,2,((#200733,#200734,#200735),(#200736,#200737,#200738),
(#200739,#200740,#200741),(#200742,#200743,#200744)),.UNSPECIFIED.,.F.,
 .F.,.F.)
B_SPLINE_SURFACE_WITH_KNOTS((4,4),(3,3),(0.,0.000397394465448312),(0.,1.),
 .UNSPECIFIED.)
GEOMETRIC_REPRESENTATION_ITEM()
RATIONAL_B_SPLINE_SURFACE(((1.,0.705498956110746,1.),(1.,0.705821764811805,
1.),(1.,0.706461952521133,1.),(1.,0.707106781186548,1.)))
REPRESENTATION_ITEM('')
SURFACE()
);
#2674=(
BOUNDED_SURFACE()
B_SPLINE_SURFACE(3,2,((#200750,#200751,#200752),(#200753,#200754,#200755),
(#200756,#200757,#200758),(#200759,#200760,#200761)),.UNSPECIFIED.,.F.,
 .F.,.F.)
B_SPLINE_SURFACE_WITH_KNOTS((4,4),(3,3),(0.,0.000397394410828737),(0.,1.),
 .UNSPECIFIED.)
GEOMETRIC_REPRESENTATION_ITEM()
RATIONAL_B_SPLINE_SURFACE(((1.,0.708689770883323,1.),(1.,0.708376440034491,
1.),(1.,0.707750498698409,1.),(1.,0.707106781186548,1.)))
REPRESENTATION_ITEM('')
SURFACE()
);
#2675=(
BOUNDED_SURFACE()
B_SPLINE_SURFACE(3,2,((#200767,#200768,#200769),(#200770,#200771,#200772),
(#200773,#200774,#200775),(#200776,#200777,#200778)),.UNSPECIFIED.,.F.,
 .F.,.F.)
B_SPLINE_SURFACE_WITH_KNOTS((4,4),(3,3),(0.,0.000511815090126173),(0.,1.00105592270387),
 .UNSPECIFIED.)
GEOMETRIC_REPRESENTATION_ITEM()
RATIONAL_B_SPLINE_SURFACE(((1.,0.705266242716999,1.00062243213183),(1.,
0.705584085908639,1.00062176089614),(1.,0.706182089450016,1.00062049800511),
(1.,0.706797508586992,1.00061919833503)))
REPRESENTATION_ITEM('')
SURFACE()
);
#2676=(
BOUNDED_SURFACE()
B_SPLINE_SURFACE(3,2,((#200780,#200781,#200782),(#200783,#200784,#200785),
(#200786,#200787,#200788),(#200789,#200790,#200791)),.UNSPECIFIED.,.F.,
 .F.,.F.)
B_SPLINE_SURFACE_WITH_KNOTS((4,4),(3,3),(0.,0.000397394428086623),(0.,1.),
 .UNSPECIFIED.)
GEOMETRIC_REPRESENTATION_ITEM()
RATIONAL_B_SPLINE_SURFACE(((1.,0.707106781186549,1.),(1.,0.706459846759093,
1.),(1.,0.70582051073728,1.),(1.,0.705498956110743,1.)))
REPRESENTATION_ITEM('')
SURFACE()
);
#2677=(
BOUNDED_SURFACE()
B_SPLINE_SURFACE(3,2,((#200797,#200798,#200799),(#200800,#200801,#200802),
(#200803,#200804,#200805),(#200806,#200807,#200808),(#200809,#200810,#200811),
(#200812,#200813,#200814)),.UNSPECIFIED.,.F.,.F.,.F.)
B_SPLINE_SURFACE_WITH_KNOTS((4,2,4),(3,3),(-1.68051336735253E-18,0.000257953807872851,
0.000515907615745705),(0.,1.),.UNSPECIFIED.)
GEOMETRIC_REPRESENTATION_ITEM()
RATIONAL_B_SPLINE_SURFACE(((1.,0.874619707139386,1.),(1.,0.874834349678948,
1.),(1.,0.854686104157841,1.),(1.,0.79247659791508,1.),(1.,0.75088785459518,
1.),(1.,0.705585838031432,1.)))
REPRESENTATION_ITEM('')
SURFACE()
);
#2678=(
BOUNDED_SURFACE()
B_SPLINE_SURFACE(3,2,((#200820,#200821,#200822),(#200823,#200824,#200825),
(#200826,#200827,#200828),(#200829,#200830,#200831)),.UNSPECIFIED.,.F.,
 .F.,.F.)
B_SPLINE_SURFACE_WITH_KNOTS((4,4),(3,3),(0.,0.000511815437699152),(0.,1.00105881331679),
 .UNSPECIFIED.)
GEOMETRIC_REPRESENTATION_ITEM()
RATIONAL_B_SPLINE_SURFACE(((1.,0.706796661946069,1.00062089519772),(1.,
0.70743082122493,1.00061955228514),(1.,0.708058545830472,1.0006182229988),
(1.,0.708394505252429,1.00061751156218)))
REPRESENTATION_ITEM('')
SURFACE()
);
#2679=(
BOUNDED_SURFACE()
B_SPLINE_SURFACE(3,2,((#200833,#200834,#200835),(#200836,#200837,#200838),
(#200839,#200840,#200841),(#200842,#200843,#200844),(#200845,#200846,#200847),
(#200848,#200849,#200850)),.UNSPECIFIED.,.F.,.F.,.F.)
B_SPLINE_SURFACE_WITH_KNOTS((4,2,4),(3,3),(-1.89735380184963E-19,0.000256915317531259,
0.000513830635062518),(0.,1.),.UNSPECIFIED.)
GEOMETRIC_REPRESENTATION_ITEM()
RATIONAL_B_SPLINE_SURFACE(((1.,0.705585838031435,1.),(1.,0.75090243354274,
1.),(1.,0.792329530082507,1.),(1.,0.854288401594194,1.),(1.,0.874998031125134,
1.),(1.,0.874619707139387,1.)))
REPRESENTATION_ITEM('')
SURFACE()
);
#2680=(
BOUNDED_SURFACE()
B_SPLINE_SURFACE(3,2,((#200856,#200857,#200858),(#200859,#200860,#200861),
(#200862,#200863,#200864),(#200865,#200866,#200867),(#200868,#200869,#200870),
(#200871,#200872,#200873)),.UNSPECIFIED.,.F.,.F.,.F.)
B_SPLINE_SURFACE_WITH_KNOTS((4,2,4),(3,3),(0.,0.000256592814262159,0.000513185628524318),
(0.,1.),.UNSPECIFIED.)
GEOMETRIC_REPRESENTATION_ITEM()
RATIONAL_B_SPLINE_SURFACE(((1.,0.708712527163674,1.),(1.,0.753780902613273,
1.),(1.,0.794538995769612,1.),(1.,0.855070770330695,1.),(1.,0.875018427445628,
1.),(1.,0.874619707139392,1.)))
REPRESENTATION_ITEM('')
SURFACE()
);
#2681=(
BOUNDED_SURFACE()
B_SPLINE_SURFACE(3,2,((#200875,#200876,#200877),(#200878,#200879,#200880),
(#200881,#200882,#200883),(#200884,#200885,#200886)),.UNSPECIFIED.,.F.,
 .F.,.F.)
B_SPLINE_SURFACE_WITH_KNOTS((4,4),(3,3),(0.,0.000511815072430392),(0.,1.00105598365776),
 .UNSPECIFIED.)
GEOMETRIC_REPRESENTATION_ITEM()
RATIONAL_B_SPLINE_SURFACE(((1.,0.70679749073401,1.0006192341164),(1.,0.706182062146944,
1.00062053388146),(1.,0.705584062769289,1.0006217968366),(1.,0.705266224770748,
1.00062246810006)))
REPRESENTATION_ITEM('')
SURFACE()
);
#2682=(
BOUNDED_SURFACE()
B_SPLINE_SURFACE(3,2,((#200892,#200893,#200894),(#200895,#200896,#200897),
(#200898,#200899,#200900),(#200901,#200902,#200903),(#200904,#200905,#200906),
(#200907,#200908,#200909)),.UNSPECIFIED.,.F.,.F.,.F.)
B_SPLINE_SURFACE_WITH_KNOTS((4,2,4),(3,3),(0.,0.000257652232350884,0.000515304464701767),
(0.,1.),.UNSPECIFIED.)
GEOMETRIC_REPRESENTATION_ITEM()
RATIONAL_B_SPLINE_SURFACE(((1.,0.87461970713939,1.),(1.,0.874861180430969,
1.),(1.,0.855455725920519,1.),(1.,0.794699358955606,1.),(1.,0.753768977788385,
1.),(1.,0.708712527163658,1.)))
REPRESENTATION_ITEM('')
SURFACE()
);
#2683=(
BOUNDED_SURFACE()
B_SPLINE_SURFACE(3,2,((#200915,#200916,#200917),(#200918,#200919,#200920),
(#200921,#200922,#200923),(#200924,#200925,#200926)),.UNSPECIFIED.,.F.,
 .F.,.F.)
B_SPLINE_SURFACE_WITH_KNOTS((4,4),(3,3),(-6.91178884959509E-18,0.000397394373651912),
(0.,1.),.UNSPECIFIED.)
GEOMETRIC_REPRESENTATION_ITEM()
RATIONAL_B_SPLINE_SURFACE(((1.,0.707106781186545,1.),(1.,0.707752587915905,
1.),(1.,0.708377654540673,1.),(1.,0.708689770883352,1.)))
REPRESENTATION_ITEM('')
SURFACE()
);
#2684=(
BOUNDED_SURFACE()
B_SPLINE_SURFACE(3,2,((#200928,#200929,#200930),(#200931,#200932,#200933),
(#200934,#200935,#200936),(#200937,#200938,#200939)),.UNSPECIFIED.,.F.,
 .F.,.F.)
B_SPLINE_SURFACE_WITH_KNOTS((4,4),(3,3),(0.,0.000511815456479794),(0.,1.00105873160034),
 .UNSPECIFIED.)
GEOMETRIC_REPRESENTATION_ITEM()
RATIONAL_B_SPLINE_SURFACE(((1.,0.708394529056221,1.00061746385384),(1.,
0.708058564166755,1.00061817524713),(1.,0.70743083537196,1.00061950443976),
(1.,0.706796685880264,1.00062084722797)))
REPRESENTATION_ITEM('')
SURFACE()
);
#2685=(
BOUNDED_SURFACE()
B_SPLINE_SURFACE(3,2,((#200945,#200946,#200947),(#200948,#200949,#200950),
(#200951,#200952,#200953),(#200954,#200955,#200956)),.UNSPECIFIED.,.F.,
 .F.,.F.)
B_SPLINE_SURFACE_WITH_KNOTS((4,4),(3,3),(-6.50521303491303E-18,0.000397394465448303),
(0.,1.),.UNSPECIFIED.)
GEOMETRIC_REPRESENTATION_ITEM()
RATIONAL_B_SPLINE_SURFACE(((1.,0.705498956110746,1.),(1.,0.705821764811771,
1.),(1.,0.70646195252114,1.),(1.,0.707106781186545,1.)))
REPRESENTATION_ITEM('')
SURFACE()
);
#2686=(
BOUNDED_SURFACE()
B_SPLINE_SURFACE(3,2,((#200962,#200963,#200964),(#200965,#200966,#200967),
(#200968,#200969,#200970),(#200971,#200972,#200973)),.UNSPECIFIED.,.F.,
 .F.,.F.)
B_SPLINE_SURFACE_WITH_KNOTS((4,4),(3,3),(0.,0.000397394410828732),(0.,1.),
 .UNSPECIFIED.)
GEOMETRIC_REPRESENTATION_ITEM()
RATIONAL_B_SPLINE_SURFACE(((1.,0.708689770883332,1.),(1.,0.708376440034489,
1.),(1.,0.707750498698412,1.),(1.,0.707106781186548,1.)))
REPRESENTATION_ITEM('')
SURFACE()
);
#2687=(
BOUNDED_SURFACE()
B_SPLINE_SURFACE(3,2,((#200979,#200980,#200981),(#200982,#200983,#200984),
(#200985,#200986,#200987),(#200988,#200989,#200990)),.UNSPECIFIED.,.F.,
 .F.,.F.)
B_SPLINE_SURFACE_WITH_KNOTS((4,4),(3,3),(0.,0.000511815090126178),(0.,1.00105592270281),
 .UNSPECIFIED.)
GEOMETRIC_REPRESENTATION_ITEM()
RATIONAL_B_SPLINE_SURFACE(((1.,0.705266242717305,1.0006224321312),(1.,0.705584085908961,
1.00062176089551),(1.,0.70618208945032,1.00062049800448),(1.,0.706797508587304,
1.0006191983344)))
REPRESENTATION_ITEM('')
SURFACE()
);
#2688=(
BOUNDED_SURFACE()
B_SPLINE_SURFACE(3,2,((#200992,#200993,#200994),(#200995,#200996,#200997),
(#200998,#200999,#201000),(#201001,#201002,#201003)),.UNSPECIFIED.,.F.,
 .F.,.F.)
B_SPLINE_SURFACE_WITH_KNOTS((4,4),(3,3),(-6.85757874097082E-18,0.00039739442808662),
(0.,1.),.UNSPECIFIED.)
GEOMETRIC_REPRESENTATION_ITEM()
RATIONAL_B_SPLINE_SURFACE(((1.,0.707106781186548,1.),(1.,0.706459846759103,
1.),(1.,0.705820510737258,1.),(1.,0.705498956110751,1.)))
REPRESENTATION_ITEM('')
SURFACE()
);
#2689=(
BOUNDED_SURFACE()
B_SPLINE_SURFACE(3,2,((#201009,#201010,#201011),(#201012,#201013,#201014),
(#201015,#201016,#201017),(#201018,#201019,#201020),(#201021,#201022,#201023),
(#201024,#201025,#201026)),.UNSPECIFIED.,.F.,.F.,.F.)
B_SPLINE_SURFACE_WITH_KNOTS((4,2,4),(3,3),(0.,0.000257953807872855,0.00051590761574571),
(0.,1.),.UNSPECIFIED.)
GEOMETRIC_REPRESENTATION_ITEM()
RATIONAL_B_SPLINE_SURFACE(((1.,0.874619707139392,1.),(1.,0.874834349678956,
1.),(1.,0.854686104157832,1.),(1.,0.79247659791509,1.),(1.,0.750887854595159,
1.),(1.,0.70558583803143,1.)))
REPRESENTATION_ITEM('')
SURFACE()
);
#2690=(
BOUNDED_SURFACE()
B_SPLINE_SURFACE(3,2,((#201032,#201033,#201034),(#201035,#201036,#201037),
(#201038,#201039,#201040),(#201041,#201042,#201043)),.UNSPECIFIED.,.F.,
 .F.,.F.)
B_SPLINE_SURFACE_WITH_KNOTS((4,4),(3,3),(0.,0.000511815437699152),(0.,1.00105881331544),
 .UNSPECIFIED.)
GEOMETRIC_REPRESENTATION_ITEM()
RATIONAL_B_SPLINE_SURFACE(((1.,0.706796661946467,1.00062089519692),(1.,
0.707430821225345,1.00061955228435),(1.,0.708058545830854,1.000618222998),
(1.,0.708394505252849,1.00061751156139)))
REPRESENTATION_ITEM('')
SURFACE()
);
#2691=(
BOUNDED_SURFACE()
B_SPLINE_SURFACE(3,2,((#201045,#201046,#201047),(#201048,#201049,#201050),
(#201051,#201052,#201053),(#201054,#201055,#201056),(#201057,#201058,#201059),
(#201060,#201061,#201062)),.UNSPECIFIED.,.F.,.F.,.F.)
B_SPLINE_SURFACE_WITH_KNOTS((4,2,4),(3,3),(-2.71050543121376E-20,0.000256915317531259,
0.000513830635062519),(0.,1.),.UNSPECIFIED.)
GEOMETRIC_REPRESENTATION_ITEM()
RATIONAL_B_SPLINE_SURFACE(((1.,0.705585838031442,1.),(1.,0.750902433542892,
1.),(1.,0.79232953008232,1.),(1.,0.854288401594389,1.),(1.,0.874998031124987,
1.),(1.,0.874619707139392,1.)))
REPRESENTATION_ITEM('')
SURFACE()
);
#2692=(
BOUNDED_SURFACE()
B_SPLINE_SURFACE(3,2,((#201068,#201069,#201070),(#201071,#201072,#201073),
(#201074,#201075,#201076),(#201077,#201078,#201079),(#201080,#201081,#201082),
(#201083,#201084,#201085)),.UNSPECIFIED.,.F.,.F.,.F.)
B_SPLINE_SURFACE_WITH_KNOTS((4,2,4),(3,3),(-9.70360944374526E-18,0.000256592814262151,
0.000513185628524312),(0.,1.),.UNSPECIFIED.)
GEOMETRIC_REPRESENTATION_ITEM()
RATIONAL_B_SPLINE_SURFACE(((1.,0.708712527163664,1.),(1.,0.753780902613591,
1.),(1.,0.79453899576919,1.),(1.,0.855070770331123,1.),(1.,0.875018427445306,
1.),(1.,0.87461970713939,1.)))
REPRESENTATION_ITEM('')
SURFACE()
);
#2693=(
BOUNDED_SURFACE()
B_SPLINE_SURFACE(3,2,((#201087,#201088,#201089),(#201090,#201091,#201092),
(#201093,#201094,#201095),(#201096,#201097,#201098)),.UNSPECIFIED.,.F.,
 .F.,.F.)
B_SPLINE_SURFACE_WITH_KNOTS((4,4),(3,3),(0.,0.000511815072430396),(0.,1.00105598365804),
 .UNSPECIFIED.)
GEOMETRIC_REPRESENTATION_ITEM()
RATIONAL_B_SPLINE_SURFACE(((1.,0.706797490733929,1.00061923411656),(1.,
0.706182062146834,1.00062053388163),(1.,0.705584062769227,1.00062179683677),
(1.,0.705266224770692,1.00062246810023)))
REPRESENTATION_ITEM('')
SURFACE()
);
#2694=(
BOUNDED_SURFACE()
B_SPLINE_SURFACE(3,2,((#201104,#201105,#201106),(#201107,#201108,#201109),
(#201110,#201111,#201112),(#201113,#201114,#201115),(#201116,#201117,#201118),
(#201119,#201120,#201121)),.UNSPECIFIED.,.F.,.F.,.F.)
B_SPLINE_SURFACE_WITH_KNOTS((4,2,4),(3,3),(-6.36968776335234E-19,0.000257652232350877,
0.000515304464701754),(0.,1.),.UNSPECIFIED.)
GEOMETRIC_REPRESENTATION_ITEM()
RATIONAL_B_SPLINE_SURFACE(((1.,0.874619707139396,1.),(1.,0.874861180430735,
1.),(1.,0.855455725920824,1.),(1.,0.794699358955301,1.),(1.,0.753768977788632,
1.),(1.,0.708712527163662,1.)))
REPRESENTATION_ITEM('')
SURFACE()
);
#2695=(
BOUNDED_SURFACE()
B_SPLINE_SURFACE(3,2,((#201127,#201128,#201129),(#201130,#201131,#201132),
(#201133,#201134,#201135),(#201136,#201137,#201138)),.UNSPECIFIED.,.F.,
 .F.,.F.)
B_SPLINE_SURFACE_WITH_KNOTS((4,4),(3,3),(0.,0.000397394373651917),(0.,1.),
 .UNSPECIFIED.)
GEOMETRIC_REPRESENTATION_ITEM()
RATIONAL_B_SPLINE_SURFACE(((1.,0.707106781186548,1.),(1.,0.70775258791587,
1.),(1.,0.708377654540717,1.),(1.,0.708689770883313,1.)))
REPRESENTATION_ITEM('')
SURFACE()
);
#2696=(
BOUNDED_SURFACE()
B_SPLINE_SURFACE(3,2,((#201140,#201141,#201142),(#201143,#201144,#201145),
(#201146,#201147,#201148),(#201149,#201150,#201151)),.UNSPECIFIED.,.F.,
 .F.,.F.)
B_SPLINE_SURFACE_WITH_KNOTS((4,4),(3,3),(0.,0.000511815456479795),(0.,1.00105873159818),
 .UNSPECIFIED.)
GEOMETRIC_REPRESENTATION_ITEM()
RATIONAL_B_SPLINE_SURFACE(((1.,0.708394529056861,1.00061746385258),(1.,
0.708058564167389,1.00061817524587),(1.,0.70743083537258,1.00061950443849),
(1.,0.706796685880899,1.0006208472267)))
REPRESENTATION_ITEM('')
SURFACE()
);
#2697=(
BOUNDED_SURFACE()
B_SPLINE_SURFACE(3,2,((#201157,#201158,#201159),(#201160,#201161,#201162),
(#201163,#201164,#201165),(#201166,#201167,#201168)),.UNSPECIFIED.,.F.,
 .F.,.F.)
B_SPLINE_SURFACE_WITH_KNOTS((4,4),(3,3),(0.,0.000397394465448298),(0.,1.),
 .UNSPECIFIED.)
GEOMETRIC_REPRESENTATION_ITEM()
RATIONAL_B_SPLINE_SURFACE(((1.,0.70549895611077,1.),(1.,0.70582176481177,
1.),(1.,0.706461952521145,1.),(1.,0.707106781186548,1.)))
REPRESENTATION_ITEM('')
SURFACE()
);
#2698=(
BOUNDED_SURFACE()
B_SPLINE_SURFACE(3,2,((#201174,#201175,#201176),(#201177,#201178,#201179),
(#201180,#201181,#201182),(#201183,#201184,#201185)),.UNSPECIFIED.,.F.,
 .F.,.F.)
B_SPLINE_SURFACE_WITH_KNOTS((4,4),(3,3),(0.,0.00039739441082875),(0.,1.),
 .UNSPECIFIED.)
GEOMETRIC_REPRESENTATION_ITEM()
RATIONAL_B_SPLINE_SURFACE(((1.,0.708689770883323,1.),(1.,0.708376440034469,
1.),(1.,0.707750498698414,1.),(1.,0.707106781186552,1.)))
REPRESENTATION_ITEM('')
SURFACE()
);
#2699=(
BOUNDED_SURFACE()
B_SPLINE_SURFACE(3,2,((#201191,#201192,#201193),(#201194,#201195,#201196),
(#201197,#201198,#201199),(#201200,#201201,#201202)),.UNSPECIFIED.,.F.,
 .F.,.F.)
B_SPLINE_SURFACE_WITH_KNOTS((4,4),(3,3),(0.,0.000511815090126182),(0.,1.00105592270276),
 .UNSPECIFIED.)
GEOMETRIC_REPRESENTATION_ITEM()
RATIONAL_B_SPLINE_SURFACE(((1.,0.705266242717327,1.00062243213117),(1.,
0.705584085908971,1.00062176089549),(1.,0.706182089450324,1.00062049800446),
(1.,0.706797508587317,1.00061919833438)))
REPRESENTATION_ITEM('')
SURFACE()
);
#2700=(
BOUNDED_SURFACE()
B_SPLINE_SURFACE(3,2,((#201204,#201205,#201206),(#201207,#201208,#201209),
(#201210,#201211,#201212),(#201213,#201214,#201215)),.UNSPECIFIED.,.F.,
 .F.,.F.)
B_SPLINE_SURFACE_WITH_KNOTS((4,4),(3,3),(0.,0.000397394428086637),(0.,1.),
 .UNSPECIFIED.)
GEOMETRIC_REPRESENTATION_ITEM()
RATIONAL_B_SPLINE_SURFACE(((1.,0.707106781186548,1.),(1.,0.706459846759089,
1.),(1.,0.705820510737281,1.),(1.,0.705498956110758,1.)))
REPRESENTATION_ITEM('')
SURFACE()
);
#2701=(
BOUNDED_SURFACE()
B_SPLINE_SURFACE(3,2,((#201221,#201222,#201223),(#201224,#201225,#201226),
(#201227,#201228,#201229),(#201230,#201231,#201232),(#201233,#201234,#201235),
(#201236,#201237,#201238)),.UNSPECIFIED.,.F.,.F.,.F.)
B_SPLINE_SURFACE_WITH_KNOTS((4,2,4),(3,3),(0.,0.000257953807872843,0.000515907615745686),
(0.,1.),.UNSPECIFIED.)
GEOMETRIC_REPRESENTATION_ITEM()
RATIONAL_B_SPLINE_SURFACE(((1.,0.874619707139388,1.),(1.,0.874834349679259,
1.),(1.,0.854686104157437,1.),(1.,0.792476597915486,1.),(1.,0.750887854594861,
1.),(1.,0.705585838031449,1.)))
REPRESENTATION_ITEM('')
SURFACE()
);
#2702=(
BOUNDED_SURFACE()
B_SPLINE_SURFACE(3,2,((#201244,#201245,#201246),(#201247,#201248,#201249),
(#201250,#201251,#201252),(#201253,#201254,#201255)),.UNSPECIFIED.,.F.,
 .F.,.F.)
B_SPLINE_SURFACE_WITH_KNOTS((4,4),(3,3),(0.,0.000511815437699153),(0.,1.00105881331748),
 .UNSPECIFIED.)
GEOMETRIC_REPRESENTATION_ITEM()
RATIONAL_B_SPLINE_SURFACE(((1.,0.706796661945868,1.00062089519812),(1.,
0.707430821224752,1.00061955228554),(1.,0.708058545830254,1.0006182229992),
(1.,0.708394505252245,1.00061751156258)))
REPRESENTATION_ITEM('')
SURFACE()
);
#2703=(
BOUNDED_SURFACE()
B_SPLINE_SURFACE(3,2,((#201257,#201258,#201259),(#201260,#201261,#201262),
(#201263,#201264,#201265),(#201266,#201267,#201268),(#201269,#201270,#201271),
(#201272,#201273,#201274)),.UNSPECIFIED.,.F.,.F.,.F.)
B_SPLINE_SURFACE_WITH_KNOTS((4,2,4),(3,3),(0.,0.000256915317531264,0.000513830635062527),
(0.,1.),.UNSPECIFIED.)
GEOMETRIC_REPRESENTATION_ITEM()
RATIONAL_B_SPLINE_SURFACE(((1.,0.705585838031439,1.),(1.,0.750902433542536,
1.),(1.,0.79232953008279,1.),(1.,0.854288401593904,1.),(1.,0.874998031125365,
1.),(1.,0.874619707139386,1.)))
REPRESENTATION_ITEM('')
SURFACE()
);
#2704=(
BOUNDED_SURFACE()
B_SPLINE_SURFACE(3,2,((#201280,#201281,#201282),(#201283,#201284,#201285),
(#201286,#201287,#201288),(#201289,#201290,#201291),(#201292,#201293,#201294),
(#201295,#201296,#201297)),.UNSPECIFIED.,.F.,.F.,.F.)
B_SPLINE_SURFACE_WITH_KNOTS((4,2,4),(3,3),(0.,0.000256592814262156,0.000513185628524312),
(0.,1.),.UNSPECIFIED.)
GEOMETRIC_REPRESENTATION_ITEM()
RATIONAL_B_SPLINE_SURFACE(((1.,0.708712527163657,1.),(1.,0.753780902613628,
1.),(1.,0.79453899576917,1.),(1.,0.85507077033114,1.),(1.,0.875018427445298,
1.),(1.,0.87461970713939,1.)))
REPRESENTATION_ITEM('')
SURFACE()
);
#2705=(
BOUNDED_SURFACE()
B_SPLINE_SURFACE(3,2,((#201299,#201300,#201301),(#201302,#201303,#201304),
(#201305,#201306,#201307),(#201308,#201309,#201310)),.UNSPECIFIED.,.F.,
 .F.,.F.)
B_SPLINE_SURFACE_WITH_KNOTS((4,4),(3,3),(2.71050543121376E-20,0.000511815072430395),
(0.,1.00105598365867),.UNSPECIFIED.)
GEOMETRIC_REPRESENTATION_ITEM()
RATIONAL_B_SPLINE_SURFACE(((1.,0.706797490733745,1.00061923411693),(1.,
0.706182062146666,1.00062053388199),(1.,0.70558406276901,1.00062179683714),
(1.,0.705266224770511,1.0006224681006)))
REPRESENTATION_ITEM('')
SURFACE()
);
#2706=(
BOUNDED_SURFACE()
B_SPLINE_SURFACE(3,2,((#201316,#201317,#201318),(#201319,#201320,#201321),
(#201322,#201323,#201324),(#201325,#201326,#201327),(#201328,#201329,#201330),
(#201331,#201332,#201333)),.UNSPECIFIED.,.F.,.F.,.F.)
B_SPLINE_SURFACE_WITH_KNOTS((4,2,4),(3,3),(0.,0.000257652232350881,0.000515304464701761),
(0.,1.),.UNSPECIFIED.)
GEOMETRIC_REPRESENTATION_ITEM()
RATIONAL_B_SPLINE_SURFACE(((1.,0.874619707139398,1.),(1.,0.874861180431049,
1.),(1.,0.855455725920415,1.),(1.,0.794699358955707,1.),(1.,0.753768977788306,
1.),(1.,0.708712527163674,1.)))
REPRESENTATION_ITEM('')
SURFACE()
);
#2707=(
BOUNDED_SURFACE()
B_SPLINE_SURFACE(3,2,((#201339,#201340,#201341),(#201342,#201343,#201344),
(#201345,#201346,#201347),(#201348,#201349,#201350)),.UNSPECIFIED.,.F.,
 .F.,.F.)
B_SPLINE_SURFACE_WITH_KNOTS((4,4),(3,3),(0.,0.000397394373651915),(0.,1.),
 .UNSPECIFIED.)
GEOMETRIC_REPRESENTATION_ITEM()
RATIONAL_B_SPLINE_SURFACE(((1.,0.707106781186548,1.),(1.,0.707752587915894,
1.),(1.,0.708377654540696,1.),(1.,0.708689770883339,1.)))
REPRESENTATION_ITEM('')
SURFACE()
);
#2708=(
BOUNDED_SURFACE()
B_SPLINE_SURFACE(3,2,((#201352,#201353,#201354),(#201355,#201356,#201357),
(#201358,#201359,#201360),(#201361,#201362,#201363)),.UNSPECIFIED.,.F.,
 .F.,.F.)
B_SPLINE_SURFACE_WITH_KNOTS((4,4),(3,3),(0.,0.000511815456479784),(0.,1.00105873159958),
 .UNSPECIFIED.)
GEOMETRIC_REPRESENTATION_ITEM()
RATIONAL_B_SPLINE_SURFACE(((1.,0.70839452905645,1.00061746385339),(1.,0.708058564166994,
1.00061817524668),(1.,0.707430835372169,1.00061950443931),(1.,0.706796685880488,
1.00062084722752)))
REPRESENTATION_ITEM('')
SURFACE()
);
#2709=(
BOUNDED_SURFACE()
B_SPLINE_SURFACE(3,2,((#201369,#201370,#201371),(#201372,#201373,#201374),
(#201375,#201376,#201377),(#201378,#201379,#201380)),.UNSPECIFIED.,.F.,
 .F.,.F.)
B_SPLINE_SURFACE_WITH_KNOTS((4,4),(3,3),(0.,0.000397394465448314),(0.,1.),
 .UNSPECIFIED.)
GEOMETRIC_REPRESENTATION_ITEM()
RATIONAL_B_SPLINE_SURFACE(((1.,0.705498956110744,1.),(1.,0.70582176481178,
1.),(1.,0.706461952521134,1.),(1.,0.707106781186548,1.)))
REPRESENTATION_ITEM('')
SURFACE()
);
#2710=(
BOUNDED_SURFACE()
B_SPLINE_SURFACE(3,2,((#201386,#201387,#201388),(#201389,#201390,#201391),
(#201392,#201393,#201394),(#201395,#201396,#201397)),.UNSPECIFIED.,.F.,
 .F.,.F.)
B_SPLINE_SURFACE_WITH_KNOTS((4,4),(3,3),(0.,0.000397394410828745),(0.,1.),
 .UNSPECIFIED.)
GEOMETRIC_REPRESENTATION_ITEM()
RATIONAL_B_SPLINE_SURFACE(((1.,0.708689770883332,1.),(1.,0.708376440034473,
1.),(1.,0.707750498698421,1.),(1.,0.707106781186548,1.)))
REPRESENTATION_ITEM('')
SURFACE()
);
#2711=(
BOUNDED_SURFACE()
B_SPLINE_SURFACE(3,2,((#201403,#201404,#201405),(#201406,#201407,#201408),
(#201409,#201410,#201411),(#201412,#201413,#201414)),.UNSPECIFIED.,.F.,
 .F.,.F.)
B_SPLINE_SURFACE_WITH_KNOTS((4,4),(3,3),(0.,0.000511815090126174),(0.,1.00105592270135),
 .UNSPECIFIED.)
GEOMETRIC_REPRESENTATION_ITEM()
RATIONAL_B_SPLINE_SURFACE(((1.,0.705266242717712,1.00062243213034),(1.,
0.705584085909422,1.00062176089466),(1.,0.706182089450735,1.00062049800363),
(1.,0.706797508587729,1.00061919833355)))
REPRESENTATION_ITEM('')
SURFACE()
);
#2712=(
BOUNDED_SURFACE()
B_SPLINE_SURFACE(3,2,((#201416,#201417,#201418),(#201419,#201420,#201421),
(#201422,#201423,#201424),(#201425,#201426,#201427)),.UNSPECIFIED.,.F.,
 .F.,.F.)
B_SPLINE_SURFACE_WITH_KNOTS((4,4),(3,3),(0.,0.00039739442808662),(0.,1.),
 .UNSPECIFIED.)
GEOMETRIC_REPRESENTATION_ITEM()
RATIONAL_B_SPLINE_SURFACE(((1.,0.707106781186552,1.),(1.,0.706459846759089,
1.),(1.,0.705820510737278,1.),(1.,0.705498956110746,1.)))
REPRESENTATION_ITEM('')
SURFACE()
);
#2713=(
BOUNDED_SURFACE()
B_SPLINE_SURFACE(3,2,((#201433,#201434,#201435),(#201436,#201437,#201438),
(#201439,#201440,#201441),(#201442,#201443,#201444),(#201445,#201446,#201447),
(#201448,#201449,#201450)),.UNSPECIFIED.,.F.,.F.,.F.)
B_SPLINE_SURFACE_WITH_KNOTS((4,2,4),(3,3),(0.,0.000257953807872838,0.000515907615745675),
(0.,1.),.UNSPECIFIED.)
GEOMETRIC_REPRESENTATION_ITEM()
RATIONAL_B_SPLINE_SURFACE(((1.,0.874619707139393,1.),(1.,0.874834349679108,
1.),(1.,0.854686104157634,1.),(1.,0.79247659791531,1.),(1.,0.75088785459499,
1.),(1.,0.70558583803147,1.)))
REPRESENTATION_ITEM('')
SURFACE()
);
#2714=(
BOUNDED_SURFACE()
B_SPLINE_SURFACE(3,2,((#201456,#201457,#201458),(#201459,#201460,#201461),
(#201462,#201463,#201464),(#201465,#201466,#201467)),.UNSPECIFIED.,.F.,
 .F.,.F.)
B_SPLINE_SURFACE_WITH_KNOTS((4,4),(3,3),(0.,0.000511815437699151),(0.,1.00105881331552),
 .UNSPECIFIED.)
GEOMETRIC_REPRESENTATION_ITEM()
RATIONAL_B_SPLINE_SURFACE(((1.,0.706796661946441,1.00062089519697),(1.,
0.707430821225319,1.0006195522844),(1.,0.708058545830829,1.00061822299806),
(1.,0.708394505252824,1.00061751156144)))
REPRESENTATION_ITEM('')
SURFACE()
);
#2715=(
BOUNDED_SURFACE()
B_SPLINE_SURFACE(3,2,((#201469,#201470,#201471),(#201472,#201473,#201474),
(#201475,#201476,#201477),(#201478,#201479,#201480),(#201481,#201482,#201483),
(#201484,#201485,#201486)),.UNSPECIFIED.,.F.,.F.,.F.)
B_SPLINE_SURFACE_WITH_KNOTS((4,2,4),(3,3),(0.,0.000256915317531257,0.000513830635062514),
(0.,1.),.UNSPECIFIED.)
GEOMETRIC_REPRESENTATION_ITEM()
RATIONAL_B_SPLINE_SURFACE(((1.,0.705585838031445,1.),(1.,0.750902433542313,
1.),(1.,0.792329530083068,1.),(1.,0.854288401593637,1.),(1.,0.874998031125529,
1.),(1.,0.874619707139391,1.)))
REPRESENTATION_ITEM('')
SURFACE()
);
#2716=(
BOUNDED_SURFACE()
B_SPLINE_SURFACE(3,2,((#201492,#201493,#201494),(#201495,#201496,#201497),
(#201498,#201499,#201500),(#201501,#201502,#201503),(#201504,#201505,#201506),
(#201507,#201508,#201509)),.UNSPECIFIED.,.F.,.F.,.F.)
B_SPLINE_SURFACE_WITH_KNOTS((4,2,4),(3,3),(0.,0.000256592814262156,0.000513185628524311),
(0.,1.),.UNSPECIFIED.)
GEOMETRIC_REPRESENTATION_ITEM()
RATIONAL_B_SPLINE_SURFACE(((1.,0.708712527163661,1.),(1.,0.753780902613512,
1.),(1.,0.794538995769294,1.),(1.,0.855070770331016,1.),(1.,0.875018427445388,
1.),(1.,0.874619707139394,1.)))
REPRESENTATION_ITEM('')
SURFACE()
);
#2717=(
BOUNDED_SURFACE()
B_SPLINE_SURFACE(3,2,((#201511,#201512,#201513),(#201514,#201515,#201516),
(#201517,#201518,#201519),(#201520,#201521,#201522)),.UNSPECIFIED.,.F.,
 .F.,.F.)
B_SPLINE_SURFACE_WITH_KNOTS((4,4),(3,3),(2.71050543121376E-20,0.000511815072430401),
(0.,1.00105598365598),.UNSPECIFIED.)
GEOMETRIC_REPRESENTATION_ITEM()
RATIONAL_B_SPLINE_SURFACE(((1.,0.706797490734529,1.00061923411535),(1.,
0.706182062147453,1.00062053388041),(1.,0.705584062769824,1.00062179683555),
(1.,0.705266224771297,1.00062246809901)))
REPRESENTATION_ITEM('')
SURFACE()
);
#2718=(
BOUNDED_SURFACE()
B_SPLINE_SURFACE(3,2,((#201528,#201529,#201530),(#201531,#201532,#201533),
(#201534,#201535,#201536),(#201537,#201538,#201539),(#201540,#201541,#201542),
(#201543,#201544,#201545)),.UNSPECIFIED.,.F.,.F.,.F.)
B_SPLINE_SURFACE_WITH_KNOTS((4,2,4),(3,3),(0.,0.000257652232350877,0.000515304464701754),
(0.,1.),.UNSPECIFIED.)
GEOMETRIC_REPRESENTATION_ITEM()
RATIONAL_B_SPLINE_SURFACE(((1.,0.874619707139384,1.),(1.,0.874861180430375,
1.),(1.,0.855455725921361,1.),(1.,0.794699358954753,1.),(1.,0.753768977789027,
1.),(1.,0.708712527163687,1.)))
REPRESENTATION_ITEM('')
SURFACE()
);
#2719=(
BOUNDED_SURFACE()
B_SPLINE_SURFACE(3,2,((#201551,#201552,#201553),(#201554,#201555,#201556),
(#201557,#201558,#201559),(#201560,#201561,#201562)),.UNSPECIFIED.,.F.,
 .F.,.F.)
B_SPLINE_SURFACE_WITH_KNOTS((4,4),(3,3),(0.,0.000397394373651915),(0.,1.),
 .UNSPECIFIED.)
GEOMETRIC_REPRESENTATION_ITEM()
RATIONAL_B_SPLINE_SURFACE(((1.,0.707106781186548,1.),(1.,0.707752587915872,
1.),(1.,0.708377654540717,1.),(1.,0.708689770883309,1.)))
REPRESENTATION_ITEM('')
SURFACE()
);
#2720=(
BOUNDED_SURFACE()
B_SPLINE_SURFACE(3,2,((#201564,#201565,#201566),(#201567,#201568,#201569),
(#201570,#201571,#201572),(#201573,#201574,#201575)),.UNSPECIFIED.,.F.,
 .F.,.F.)
B_SPLINE_SURFACE_WITH_KNOTS((4,4),(3,3),(0.,0.000511815456479786),(0.,1.00105873159942),
 .UNSPECIFIED.)
GEOMETRIC_REPRESENTATION_ITEM()
RATIONAL_B_SPLINE_SURFACE(((1.,0.708394529056477,1.0006174638533),(1.,0.70805856416704,
1.00061817524659),(1.,0.70743083537222,1.00061950443921),(1.,0.706796685880534,
1.00062084722743)))
REPRESENTATION_ITEM('')
SURFACE()
);
#2721=(
BOUNDED_SURFACE()
B_SPLINE_SURFACE(3,2,((#201581,#201582,#201583),(#201584,#201585,#201586),
(#201587,#201588,#201589),(#201590,#201591,#201592)),.UNSPECIFIED.,.F.,
 .F.,.F.)
B_SPLINE_SURFACE_WITH_KNOTS((4,4),(3,3),(0.,0.000397394465448303),(0.,1.),
 .UNSPECIFIED.)
GEOMETRIC_REPRESENTATION_ITEM()
RATIONAL_B_SPLINE_SURFACE(((1.,0.705498956110749,1.),(1.,0.705821764811794,
1.),(1.,0.706461952521135,1.),(1.,0.707106781186552,1.)))
REPRESENTATION_ITEM('')
SURFACE()
);
#2722=(
BOUNDED_SURFACE()
B_SPLINE_SURFACE(3,2,((#201598,#201599,#201600),(#201601,#201602,#201603),
(#201604,#201605,#201606),(#201607,#201608,#201609)),.UNSPECIFIED.,.F.,
 .F.,.F.)
B_SPLINE_SURFACE_WITH_KNOTS((4,4),(3,3),(0.,0.000397394410828744),(0.,1.),
 .UNSPECIFIED.)
GEOMETRIC_REPRESENTATION_ITEM()
RATIONAL_B_SPLINE_SURFACE(((1.,0.708689770883327,1.),(1.,0.708376440034467,
1.),(1.,0.707750498698417,1.),(1.,0.707106781186553,1.)))
REPRESENTATION_ITEM('')
SURFACE()
);
#2723=(
BOUNDED_SURFACE()
B_SPLINE_SURFACE(3,2,((#201615,#201616,#201617),(#201618,#201619,#201620),
(#201621,#201622,#201623),(#201624,#201625,#201626)),.UNSPECIFIED.,.F.,
 .F.,.F.)
B_SPLINE_SURFACE_WITH_KNOTS((4,4),(3,3),(0.,0.000511815090126171),(0.,1.00105592270426),
 .UNSPECIFIED.)
GEOMETRIC_REPRESENTATION_ITEM()
RATIONAL_B_SPLINE_SURFACE(((1.,0.705266242716881,1.00062243213206),(1.,
0.70558408590855,1.00062176089637),(1.,0.706182089449876,1.00062049800534),
(1.,0.706797508586871,1.00061919833526)))
REPRESENTATION_ITEM('')
SURFACE()
);
#2724=(
BOUNDED_SURFACE()
B_SPLINE_SURFACE(3,2,((#201628,#201629,#201630),(#201631,#201632,#201633),
(#201634,#201635,#201636),(#201637,#201638,#201639)),.UNSPECIFIED.,.F.,
 .F.,.F.)
B_SPLINE_SURFACE_WITH_KNOTS((4,4),(3,3),(0.,0.000397394428086638),(0.,1.),
 .UNSPECIFIED.)
GEOMETRIC_REPRESENTATION_ITEM()
RATIONAL_B_SPLINE_SURFACE(((1.,0.707106781186542,1.),(1.,0.706459846759111,
1.),(1.,0.705820510737245,1.),(1.,0.705498956110775,1.)))
REPRESENTATION_ITEM('')
SURFACE()
);
#2725=(
BOUNDED_SURFACE()
B_SPLINE_SURFACE(3,2,((#201645,#201646,#201647),(#201648,#201649,#201650),
(#201651,#201652,#201653),(#201654,#201655,#201656),(#201657,#201658,#201659),
(#201660,#201661,#201662)),.UNSPECIFIED.,.F.,.F.,.F.)
B_SPLINE_SURFACE_WITH_KNOTS((4,2,4),(3,3),(0.,0.000257953807872846,0.000515907615745693),
(0.,1.),.UNSPECIFIED.)
GEOMETRIC_REPRESENTATION_ITEM()
RATIONAL_B_SPLINE_SURFACE(((1.,0.874619707139392,1.),(1.,0.874834349678654,
1.),(1.,0.854686104158254,1.),(1.,0.792476597914678,1.),(1.,0.750887854595472,
1.),(1.,0.705585838031445,1.)))
REPRESENTATION_ITEM('')
SURFACE()
);
#2726=(
BOUNDED_SURFACE()
B_SPLINE_SURFACE(3,2,((#201668,#201669,#201670),(#201671,#201672,#201673),
(#201674,#201675,#201676),(#201677,#201678,#201679)),.UNSPECIFIED.,.F.,
 .F.,.F.)
B_SPLINE_SURFACE_WITH_KNOTS((4,4),(3,3),(0.,0.000511815437699147),(0.,1.00105881331846),
 .UNSPECIFIED.)
GEOMETRIC_REPRESENTATION_ITEM()
RATIONAL_B_SPLINE_SURFACE(((1.,0.706796661945576,1.0006208951987),(1.,0.707430821224465,
1.00061955228611),(1.,0.708058545829957,1.00061822299977),(1.,0.708394505251969,
1.00061751156315)))
REPRESENTATION_ITEM('')
SURFACE()
);
#2727=(
BOUNDED_SURFACE()
B_SPLINE_SURFACE(3,2,((#201681,#201682,#201683),(#201684,#201685,#201686),
(#201687,#201688,#201689),(#201690,#201691,#201692),(#201693,#201694,#201695),
(#201696,#201697,#201698)),.UNSPECIFIED.,.F.,.F.,.F.)
B_SPLINE_SURFACE_WITH_KNOTS((4,2,4),(3,3),(0.,0.00025691531753127,0.00051383063506254),
(0.,1.),.UNSPECIFIED.)
GEOMETRIC_REPRESENTATION_ITEM()
RATIONAL_B_SPLINE_SURFACE(((1.,0.705585838031441,1.),(1.,0.750902433542855,
1.),(1.,0.792329530082382,1.),(1.,0.854288401594348,1.),(1.,0.874998031125036,
1.),(1.,0.874619707139405,1.)))
REPRESENTATION_ITEM('')
SURFACE()
);
#2728=(
BOUNDED_SURFACE()
B_SPLINE_SURFACE(3,2,((#201704,#201705,#201706),(#201707,#201708,#201709),
(#201710,#201711,#201712),(#201713,#201714,#201715),(#201716,#201717,#201718),
(#201719,#201720,#201721)),.UNSPECIFIED.,.F.,.F.,.F.)
B_SPLINE_SURFACE_WITH_KNOTS((4,2,4),(3,3),(-5.77337656848531E-18,0.000256592814262152,
0.00051318562852431),(0.,1.),.UNSPECIFIED.)
GEOMETRIC_REPRESENTATION_ITEM()
RATIONAL_B_SPLINE_SURFACE(((1.,0.708712527163657,1.),(1.,0.753780902613262,
1.),(1.,0.794538995769635,1.),(1.,0.855070770330661,1.),(1.,0.875018427445639,
1.),(1.,0.874619707139395,1.)))
REPRESENTATION_ITEM('')
SURFACE()
);
#2729=(
BOUNDED_SURFACE()
B_SPLINE_SURFACE(3,2,((#201723,#201724,#201725),(#201726,#201727,#201728),
(#201729,#201730,#201731),(#201732,#201733,#201734)),.UNSPECIFIED.,.F.,
 .F.,.F.)
B_SPLINE_SURFACE_WITH_KNOTS((4,4),(3,3),(0.,0.000511815072430395),(0.,1.00105598366015),
 .UNSPECIFIED.)
GEOMETRIC_REPRESENTATION_ITEM()
RATIONAL_B_SPLINE_SURFACE(((1.,0.706797490733319,1.0006192341178),(1.,0.706182062146218,
1.00062053388286),(1.,0.705584062768601,1.00062179683801),(1.,0.705266224770064,
1.00062246810147)))
REPRESENTATION_ITEM('')
SURFACE()
);
#2730=(
BOUNDED_SURFACE()
B_SPLINE_SURFACE(3,2,((#201740,#201741,#201742),(#201743,#201744,#201745),
(#201746,#201747,#201748),(#201749,#201750,#201751),(#201752,#201753,#201754),
(#201755,#201756,#201757)),.UNSPECIFIED.,.F.,.F.,.F.)
B_SPLINE_SURFACE_WITH_KNOTS((4,2,4),(3,3),(-3.36102673470506E-18,0.000257652232350881,
0.000515304464701766),(0.,1.),.UNSPECIFIED.)
GEOMETRIC_REPRESENTATION_ITEM()
RATIONAL_B_SPLINE_SURFACE(((1.,0.874619707139375,1.),(1.,0.874861180430626,
1.),(1.,0.855455725920945,1.),(1.,0.79469935895517,1.),(1.,0.753768977788711,
1.),(1.,0.708712527163638,1.)))
REPRESENTATION_ITEM('')
SURFACE()
);
#2731=(
BOUNDED_SURFACE()
B_SPLINE_SURFACE(3,2,((#201763,#201764,#201765),(#201766,#201767,#201768),
(#201769,#201770,#201771),(#201772,#201773,#201774)),.UNSPECIFIED.,.F.,
 .F.,.F.)
B_SPLINE_SURFACE_WITH_KNOTS((4,4),(3,3),(0.,0.000397394373651913),(0.,1.),
 .UNSPECIFIED.)
GEOMETRIC_REPRESENTATION_ITEM()
RATIONAL_B_SPLINE_SURFACE(((1.,0.707106781186548,1.),(1.,0.707752587915885,
1.),(1.,0.708377654540686,1.),(1.,0.708689770883335,1.)))
REPRESENTATION_ITEM('')
SURFACE()
);
#2732=(
BOUNDED_SURFACE()
B_SPLINE_SURFACE(3,2,((#201776,#201777,#201778),(#201779,#201780,#201781),
(#201782,#201783,#201784),(#201785,#201786,#201787)),.UNSPECIFIED.,.F.,
 .F.,.F.)
B_SPLINE_SURFACE_WITH_KNOTS((4,4),(3,3),(0.,0.000511815456479783),(0.,1.00105873160181),
 .UNSPECIFIED.)
GEOMETRIC_REPRESENTATION_ITEM()
RATIONAL_B_SPLINE_SURFACE(((1.,0.708394529055794,1.0006174638547),(1.,0.708058564166318,
1.00061817524799),(1.,0.707430835371533,1.00061950444062),(1.,0.706796685879833,
1.00062084722883)))
REPRESENTATION_ITEM('')
SURFACE()
);
#2733=(
BOUNDED_SURFACE()
B_SPLINE_SURFACE(3,2,((#201793,#201794,#201795),(#201796,#201797,#201798),
(#201799,#201800,#201801),(#201802,#201803,#201804)),.UNSPECIFIED.,.F.,
 .F.,.F.)
B_SPLINE_SURFACE_WITH_KNOTS((4,4),(3,3),(0.,0.000397394465448324),(0.,1.),
 .UNSPECIFIED.)
GEOMETRIC_REPRESENTATION_ITEM()
RATIONAL_B_SPLINE_SURFACE(((1.,0.705498956110748,1.),(1.,0.70582176481177,
1.),(1.,0.706461952521139,1.),(1.,0.707106781186553,1.)))
REPRESENTATION_ITEM('')
SURFACE()
);
#2734=(
BOUNDED_SURFACE()
B_SPLINE_SURFACE(3,2,((#201810,#201811,#201812),(#201813,#201814,#201815),
(#201816,#201817,#201818),(#201819,#201820,#201821)),.UNSPECIFIED.,.F.,
 .F.,.F.)
B_SPLINE_SURFACE_WITH_KNOTS((4,4),(3,3),(0.,0.000397394410828724),(0.,1.),
 .UNSPECIFIED.)
GEOMETRIC_REPRESENTATION_ITEM()
RATIONAL_B_SPLINE_SURFACE(((1.,0.708689770883328,1.),(1.,0.708376440034509,
1.),(1.,0.707750498698382,1.),(1.,0.707106781186548,1.)))
REPRESENTATION_ITEM('')
SURFACE()
);
#2735=(
BOUNDED_SURFACE()
B_SPLINE_SURFACE(3,2,((#201827,#201828,#201829),(#201830,#201831,#201832),
(#201833,#201834,#201835),(#201836,#201837,#201838)),.UNSPECIFIED.,.F.,
 .F.,.F.)
B_SPLINE_SURFACE_WITH_KNOTS((4,4),(3,3),(0.,0.000511815090126181),(0.,1.00105592270307),
 .UNSPECIFIED.)
GEOMETRIC_REPRESENTATION_ITEM()
RATIONAL_B_SPLINE_SURFACE(((1.,0.70526624271723,1.00062243213135),(1.,0.705584085908917,
1.00062176089567),(1.,0.706182089450198,1.00062049800464),(1.,0.706797508587235,
1.00061919833456)))
REPRESENTATION_ITEM('')
SURFACE()
);
#2736=(
BOUNDED_SURFACE()
B_SPLINE_SURFACE(3,2,((#201840,#201841,#201842),(#201843,#201844,#201845),
(#201846,#201847,#201848),(#201849,#201850,#201851)),.UNSPECIFIED.,.F.,
 .F.,.F.)
B_SPLINE_SURFACE_WITH_KNOTS((4,4),(3,3),(0.,0.000397394428086613),(0.,1.),
 .UNSPECIFIED.)
GEOMETRIC_REPRESENTATION_ITEM()
RATIONAL_B_SPLINE_SURFACE(((1.,0.707106781186548,1.),(1.,0.706459846759089,
1.),(1.,0.70582051073727,1.),(1.,0.705498956110753,1.)))
REPRESENTATION_ITEM('')
SURFACE()
);
#2737=(
BOUNDED_SURFACE()
B_SPLINE_SURFACE(3,2,((#201857,#201858,#201859),(#201860,#201861,#201862),
(#201863,#201864,#201865),(#201866,#201867,#201868),(#201869,#201870,#201871),
(#201872,#201873,#201874)),.UNSPECIFIED.,.F.,.F.,.F.)
B_SPLINE_SURFACE_WITH_KNOTS((4,2,4),(3,3),(0.,0.000257953807872844,0.000515907615745687),
(0.,1.),.UNSPECIFIED.)
GEOMETRIC_REPRESENTATION_ITEM()
RATIONAL_B_SPLINE_SURFACE(((1.,0.874619707139387,1.),(1.,0.874834349679082,
1.),(1.,0.854686104157689,1.),(1.,0.792476597915248,1.),(1.,0.750887854595037,
1.),(1.,0.70558583803144,1.)))
REPRESENTATION_ITEM('')
SURFACE()
);
#2738=(
BOUNDED_SURFACE()
B_SPLINE_SURFACE(3,2,((#201880,#201881,#201882),(#201883,#201884,#201885),
(#201886,#201887,#201888),(#201889,#201890,#201891)),.UNSPECIFIED.,.F.,
 .F.,.F.)
B_SPLINE_SURFACE_WITH_KNOTS((4,4),(3,3),(0.,0.000511815437699158),(0.,1.00105881331624),
 .UNSPECIFIED.)
GEOMETRIC_REPRESENTATION_ITEM()
RATIONAL_B_SPLINE_SURFACE(((1.,0.706796661946222,1.0006208951974),(1.,0.707430821225124,
1.00061955228482),(1.,0.708058545830611,1.00061822299848),(1.,0.708394505252608,
1.00061751156186)))
REPRESENTATION_ITEM('')
SURFACE()
);
#2739=(
BOUNDED_SURFACE()
B_SPLINE_SURFACE(3,2,((#201893,#201894,#201895),(#201896,#201897,#201898),
(#201899,#201900,#201901),(#201902,#201903,#201904),(#201905,#201906,#201907),
(#201908,#201909,#201910)),.UNSPECIFIED.,.F.,.F.,.F.)
B_SPLINE_SURFACE_WITH_KNOTS((4,2,4),(3,3),(0.,0.00025691531753126,0.00051383063506252),
(0.,1.),.UNSPECIFIED.)
GEOMETRIC_REPRESENTATION_ITEM()
RATIONAL_B_SPLINE_SURFACE(((1.,0.705585838031443,1.),(1.,0.750902433542485,
1.),(1.,0.792329530082859,1.),(1.,0.854288401593878,1.),(1.,0.874998031125374,
1.),(1.,0.874619707139411,1.)))
REPRESENTATION_ITEM('')
SURFACE()
);
#2740=(
BOUNDED_SURFACE()
B_SPLINE_SURFACE(3,2,((#201916,#201917,#201918),(#201919,#201920,#201921),
(#201922,#201923,#201924),(#201925,#201926,#201927),(#201928,#201929,#201930),
(#201931,#201932,#201933)),.UNSPECIFIED.,.F.,.F.,.F.)
B_SPLINE_SURFACE_WITH_KNOTS((4,2,4),(3,3),(0.,0.000256592814262158,0.000513185628524317),
(0.,1.),.UNSPECIFIED.)
GEOMETRIC_REPRESENTATION_ITEM()
RATIONAL_B_SPLINE_SURFACE(((1.,0.708712527163662,1.),(1.,0.753780902613653,
1.),(1.,0.794538995769098,1.),(1.,0.855070770331221,1.),(1.,0.875018427445238,
1.),(1.,0.874619707139383,1.)))
REPRESENTATION_ITEM('')
SURFACE()
);
#2741=(
BOUNDED_SURFACE()
B_SPLINE_SURFACE(3,2,((#201935,#201936,#201937),(#201938,#201939,#201940),
(#201941,#201942,#201943),(#201944,#201945,#201946)),.UNSPECIFIED.,.F.,
 .F.,.F.)
B_SPLINE_SURFACE_WITH_KNOTS((4,4),(3,3),(2.71050543121376E-20,0.000511815072430396),
(0.,1.00105598366068),.UNSPECIFIED.)
GEOMETRIC_REPRESENTATION_ITEM()
RATIONAL_B_SPLINE_SURFACE(((1.,0.706797490733148,1.00061923411811),(1.,
0.706182062146073,1.00062053388318),(1.,0.705584062768447,1.00062179683832),
(1.,0.705266224769915,1.00062246810179)))
REPRESENTATION_ITEM('')
SURFACE()
);
#2742=(
BOUNDED_SURFACE()
B_SPLINE_SURFACE(3,2,((#201952,#201953,#201954),(#201955,#201956,#201957),
(#201958,#201959,#201960),(#201961,#201962,#201963),(#201964,#201965,#201966),
(#201967,#201968,#201969)),.UNSPECIFIED.,.F.,.F.,.F.)
B_SPLINE_SURFACE_WITH_KNOTS((4,2,4),(3,3),(0.,0.000257652232350886,0.000515304464701772),
(0.,1.),.UNSPECIFIED.)
GEOMETRIC_REPRESENTATION_ITEM()
RATIONAL_B_SPLINE_SURFACE(((1.,0.87461970713939,1.),(1.,0.874861180430661,
1.),(1.,0.855455725920899,1.),(1.,0.794699358955201,1.),(1.,0.753768977788728,
1.),(1.,0.708712527163643,1.)))
REPRESENTATION_ITEM('')
SURFACE()
);
#2743=(
BOUNDED_SURFACE()
B_SPLINE_SURFACE(3,2,((#201975,#201976,#201977),(#201978,#201979,#201980),
(#201981,#201982,#201983),(#201984,#201985,#201986)),.UNSPECIFIED.,.F.,
 .F.,.F.)
B_SPLINE_SURFACE_WITH_KNOTS((4,4),(3,3),(0.,0.000397394373651917),(0.,1.),
 .UNSPECIFIED.)
GEOMETRIC_REPRESENTATION_ITEM()
RATIONAL_B_SPLINE_SURFACE(((1.,0.707106781186548,1.),(1.,0.70775258791592,
1.),(1.,0.708377654540679,1.),(1.,0.708689770883336,1.)))
REPRESENTATION_ITEM('')
SURFACE()
);
#2744=(
BOUNDED_SURFACE()
B_SPLINE_SURFACE(3,2,((#201988,#201989,#201990),(#201991,#201992,#201993),
(#201994,#201995,#201996),(#201997,#201998,#201999)),.UNSPECIFIED.,.F.,
 .F.,.F.)
B_SPLINE_SURFACE_WITH_KNOTS((4,4),(3,3),(0.,0.000511815456479786),(0.,1.00105873160188),
 .UNSPECIFIED.)
GEOMETRIC_REPRESENTATION_ITEM()
RATIONAL_B_SPLINE_SURFACE(((1.,0.708394529055777,1.00061746385474),(1.,
0.708058564166309,1.00061817524803),(1.,0.707430835371485,1.00061950444066),
(1.,0.706796685879812,1.00062084722887)))
REPRESENTATION_ITEM('')
SURFACE()
);
#2745=(
BOUNDED_SURFACE()
B_SPLINE_SURFACE(3,2,((#202005,#202006,#202007),(#202008,#202009,#202010),
(#202011,#202012,#202013),(#202014,#202015,#202016)),.UNSPECIFIED.,.F.,
 .F.,.F.)
B_SPLINE_SURFACE_WITH_KNOTS((4,4),(3,3),(0.,0.000397394465448299),(0.,1.),
 .UNSPECIFIED.)
GEOMETRIC_REPRESENTATION_ITEM()
RATIONAL_B_SPLINE_SURFACE(((1.,0.70549895611075,1.),(1.,0.705821764811771,
1.),(1.,0.70646195252116,1.),(1.,0.707106781186548,1.)))
REPRESENTATION_ITEM('')
SURFACE()
);
#2746=(
BOUNDED_SURFACE()
B_SPLINE_SURFACE(3,2,((#202022,#202023,#202024),(#202025,#202026,#202027),
(#202028,#202029,#202030),(#202031,#202032,#202033)),.UNSPECIFIED.,.F.,
 .F.,.F.)
B_SPLINE_SURFACE_WITH_KNOTS((4,4),(3,3),(0.,0.000397394410828727),(0.,1.),
 .UNSPECIFIED.)
GEOMETRIC_REPRESENTATION_ITEM()
RATIONAL_B_SPLINE_SURFACE(((1.,0.708689770883334,1.),(1.,0.708376440034467,
1.),(1.,0.707750498698424,1.),(1.,0.707106781186538,1.)))
REPRESENTATION_ITEM('')
SURFACE()
);
#2747=(
BOUNDED_SURFACE()
B_SPLINE_SURFACE(3,2,((#202039,#202040,#202041),(#202042,#202043,#202044),
(#202045,#202046,#202047),(#202048,#202049,#202050)),.UNSPECIFIED.,.F.,
 .F.,.F.)
B_SPLINE_SURFACE_WITH_KNOTS((4,4),(3,3),(0.,0.000511815090126184),(0.,1.00105592270359),
 .UNSPECIFIED.)
GEOMETRIC_REPRESENTATION_ITEM()
RATIONAL_B_SPLINE_SURFACE(((1.,0.705266242717073,1.00062243213166),(1.,
0.70558408590872,1.00062176089597),(1.,0.706182089450093,1.00062049800494),
(1.,0.706797508587065,1.00061919833486)))
REPRESENTATION_ITEM('')
SURFACE()
);
#2748=(
BOUNDED_SURFACE()
B_SPLINE_SURFACE(3,2,((#202052,#202053,#202054),(#202055,#202056,#202057),
(#202058,#202059,#202060),(#202061,#202062,#202063)),.UNSPECIFIED.,.F.,
 .F.,.F.)
B_SPLINE_SURFACE_WITH_KNOTS((4,4),(3,3),(0.,0.00039739442808662),(0.,1.),
 .UNSPECIFIED.)
GEOMETRIC_REPRESENTATION_ITEM()
RATIONAL_B_SPLINE_SURFACE(((1.,0.707106781186548,1.),(1.,0.706459846759105,
1.),(1.,0.705820510737281,1.),(1.,0.705498956110749,1.)))
REPRESENTATION_ITEM('')
SURFACE()
);
#2749=(
BOUNDED_SURFACE()
B_SPLINE_SURFACE(3,2,((#202069,#202070,#202071),(#202072,#202073,#202074),
(#202075,#202076,#202077),(#202078,#202079,#202080),(#202081,#202082,#202083),
(#202084,#202085,#202086)),.UNSPECIFIED.,.F.,.F.,.F.)
B_SPLINE_SURFACE_WITH_KNOTS((4,2,4),(3,3),(0.,0.000257953807872843,0.000515907615745687),
(0.,1.),.UNSPECIFIED.)
GEOMETRIC_REPRESENTATION_ITEM()
RATIONAL_B_SPLINE_SURFACE(((1.,0.874619707139391,1.),(1.,0.874834349679335,
1.),(1.,0.854686104157323,1.),(1.,0.792476597915613,1.),(1.,0.750887854594751,
1.),(1.,0.705585838031461,1.)))
REPRESENTATION_ITEM('')
SURFACE()
);
#2750=(
BOUNDED_SURFACE()
B_SPLINE_SURFACE(3,2,((#202092,#202093,#202094),(#202095,#202096,#202097),
(#202098,#202099,#202100),(#202101,#202102,#202103)),.UNSPECIFIED.,.F.,
 .F.,.F.)
B_SPLINE_SURFACE_WITH_KNOTS((4,4),(3,3),(0.,0.000511815437699148),(0.,1.00105881332022),
 .UNSPECIFIED.)
GEOMETRIC_REPRESENTATION_ITEM()
RATIONAL_B_SPLINE_SURFACE(((1.,0.706796661945066,1.00062089519973),(1.,
0.707430821223953,1.00061955228715),(1.,0.708058545829438,1.0006182230008),
(1.,0.70839450525146,1.00061751156418)))
REPRESENTATION_ITEM('')
SURFACE()
);
#2751=(
BOUNDED_SURFACE()
B_SPLINE_SURFACE(3,2,((#202105,#202106,#202107),(#202108,#202109,#202110),
(#202111,#202112,#202113),(#202114,#202115,#202116),(#202117,#202118,#202119),
(#202120,#202121,#202122)),.UNSPECIFIED.,.F.,.F.,.F.)
B_SPLINE_SURFACE_WITH_KNOTS((4,2,4),(3,3),(0.,0.00025691531753126,0.00051383063506252),
(0.,1.),.UNSPECIFIED.)
GEOMETRIC_REPRESENTATION_ITEM()
RATIONAL_B_SPLINE_SURFACE(((1.,0.705585838031456,1.),(1.,0.750902433542557,
1.),(1.,0.792329530082758,1.),(1.,0.854288401593967,1.),(1.,0.874998031125322,
1.),(1.,0.874619707139389,1.)))
REPRESENTATION_ITEM('')
SURFACE()
);
#2752=(
BOUNDED_SURFACE()
B_SPLINE_SURFACE(3,2,((#202128,#202129,#202130),(#202131,#202132,#202133),
(#202134,#202135,#202136),(#202137,#202138,#202139),(#202140,#202141,#202142),
(#202143,#202144,#202145)),.UNSPECIFIED.,.F.,.F.,.F.)
B_SPLINE_SURFACE_WITH_KNOTS((4,2,4),(3,3),(0.,0.000256592814262157,0.000513185628524313),
(0.,1.),.UNSPECIFIED.)
GEOMETRIC_REPRESENTATION_ITEM()
RATIONAL_B_SPLINE_SURFACE(((1.,0.708712527163664,1.),(1.,0.753780902613438,
1.),(1.,0.794538995769409,1.),(1.,0.855070770330893,1.),(1.,0.87501842744548,
1.),(1.,0.874619707139388,1.)))
REPRESENTATION_ITEM('')
SURFACE()
);
#2753=(
BOUNDED_SURFACE()
B_SPLINE_SURFACE(3,2,((#202147,#202148,#202149),(#202150,#202151,#202152),
(#202153,#202154,#202155),(#202156,#202157,#202158)),.UNSPECIFIED.,.F.,
 .F.,.F.)
B_SPLINE_SURFACE_WITH_KNOTS((4,4),(3,3),(0.,0.000511815072430396),(0.,1.001055983657),
 .UNSPECIFIED.)
GEOMETRIC_REPRESENTATION_ITEM()
RATIONAL_B_SPLINE_SURFACE(((1.,0.706797490734233,1.00061923411595),(1.,
0.706182062147162,1.00062053388101),(1.,0.705584062769501,1.00062179683615),
(1.,0.705266224770988,1.00062246809962)))
REPRESENTATION_ITEM('')
SURFACE()
);
#2754=(
BOUNDED_SURFACE()
B_SPLINE_SURFACE(3,2,((#202164,#202165,#202166),(#202167,#202168,#202169),
(#202170,#202171,#202172),(#202173,#202174,#202175),(#202176,#202177,#202178),
(#202179,#202180,#202181)),.UNSPECIFIED.,.F.,.F.,.F.)
B_SPLINE_SURFACE_WITH_KNOTS((4,2,4),(3,3),(-3.10352871873976E-18,0.00025765223235088,
0.000515304464701763),(0.,1.),.UNSPECIFIED.)
GEOMETRIC_REPRESENTATION_ITEM()
RATIONAL_B_SPLINE_SURFACE(((1.,0.874619707139394,1.),(1.,0.874861180430981,
1.),(1.,0.855455725920473,1.),(1.,0.794699358955668,1.),(1.,0.753768977788342,
1.),(1.,0.708712527163659,1.)))
REPRESENTATION_ITEM('')
SURFACE()
);
#2755=(
BOUNDED_SURFACE()
B_SPLINE_SURFACE(3,2,((#202187,#202188,#202189),(#202190,#202191,#202192),
(#202193,#202194,#202195),(#202196,#202197,#202198)),.UNSPECIFIED.,.F.,
 .F.,.F.)
B_SPLINE_SURFACE_WITH_KNOTS((4,4),(3,3),(2.71050543121376E-20,0.000397394373651914),
(0.,1.),.UNSPECIFIED.)
GEOMETRIC_REPRESENTATION_ITEM()
RATIONAL_B_SPLINE_SURFACE(((1.,0.707106781186538,1.),(1.,0.707752587915903,
1.),(1.,0.708377654540675,1.),(1.,0.708689770883326,1.)))
REPRESENTATION_ITEM('')
SURFACE()
);
#2756=(
BOUNDED_SURFACE()
B_SPLINE_SURFACE(3,2,((#202200,#202201,#202202),(#202203,#202204,#202205),
(#202206,#202207,#202208),(#202209,#202210,#202211)),.UNSPECIFIED.,.F.,
 .F.,.F.)
B_SPLINE_SURFACE_WITH_KNOTS((4,4),(3,3),(0.,0.000511815456479788),(0.,1.00105873159876),
 .UNSPECIFIED.)
GEOMETRIC_REPRESENTATION_ITEM()
RATIONAL_B_SPLINE_SURFACE(((1.,0.708394529056676,1.00061746385292),(1.,
0.708058564167226,1.00061817524621),(1.,0.707430835372413,1.00061950443883),
(1.,0.706796685880726,1.00062084722704)))
REPRESENTATION_ITEM('')
SURFACE()
);
#2757=(
BOUNDED_SURFACE()
B_SPLINE_SURFACE(3,2,((#202217,#202218,#202219),(#202220,#202221,#202222),
(#202223,#202224,#202225),(#202226,#202227,#202228)),.UNSPECIFIED.,.F.,
 .F.,.F.)
B_SPLINE_SURFACE_WITH_KNOTS((4,4),(3,3),(0.,0.000397394465448322),(0.,1.),
 .UNSPECIFIED.)
GEOMETRIC_REPRESENTATION_ITEM()
RATIONAL_B_SPLINE_SURFACE(((1.,0.705498956110748,1.),(1.,0.705821764811803,
1.),(1.,0.706461952521134,1.),(1.,0.707106781186529,1.)))
REPRESENTATION_ITEM('')
SURFACE()
);
#2758=(
BOUNDED_SURFACE()
B_SPLINE_SURFACE(3,2,((#202234,#202235,#202236),(#202237,#202238,#202239),
(#202240,#202241,#202242),(#202243,#202244,#202245)),.UNSPECIFIED.,.F.,
 .F.,.F.)
B_SPLINE_SURFACE_WITH_KNOTS((4,4),(3,3),(0.,0.00039739441082874),(0.,1.),
 .UNSPECIFIED.)
GEOMETRIC_REPRESENTATION_ITEM()
RATIONAL_B_SPLINE_SURFACE(((1.,0.708689770883322,1.),(1.,0.708376440034495,
1.),(1.,0.707750498698404,1.),(1.,0.707106781186548,1.)))
REPRESENTATION_ITEM('')
SURFACE()
);
#2759=(
BOUNDED_SURFACE()
B_SPLINE_SURFACE(3,2,((#202251,#202252,#202253),(#202254,#202255,#202256),
(#202257,#202258,#202259),(#202260,#202261,#202262)),.UNSPECIFIED.,.F.,
 .F.,.F.)
B_SPLINE_SURFACE_WITH_KNOTS((4,4),(3,3),(0.,0.000511815090126184),(0.,1.00105592270412),
 .UNSPECIFIED.)
GEOMETRIC_REPRESENTATION_ITEM()
RATIONAL_B_SPLINE_SURFACE(((1.,0.705266242716956,1.00062243213197),(1.,
0.705584085908522,1.00062176089629),(1.,0.706182089449954,1.00062049800525),
(1.,0.706797508586919,1.00061919833518)))
REPRESENTATION_ITEM('')
SURFACE()
);
#2760=(
BOUNDED_SURFACE()
B_SPLINE_SURFACE(3,2,((#202264,#202265,#202266),(#202267,#202268,#202269),
(#202270,#202271,#202272),(#202273,#202274,#202275)),.UNSPECIFIED.,.F.,
 .F.,.F.)
B_SPLINE_SURFACE_WITH_KNOTS((4,4),(3,3),(0.,0.000397394428086625),(0.,1.),
 .UNSPECIFIED.)
GEOMETRIC_REPRESENTATION_ITEM()
RATIONAL_B_SPLINE_SURFACE(((1.,0.707106781186548,1.),(1.,0.706459846759129,
1.),(1.,0.705820510737238,1.),(1.,0.705498956110761,1.)))
REPRESENTATION_ITEM('')
SURFACE()
);
#2761=(
BOUNDED_SURFACE()
B_SPLINE_SURFACE(3,2,((#202281,#202282,#202283),(#202284,#202285,#202286),
(#202287,#202288,#202289),(#202290,#202291,#202292),(#202293,#202294,#202295),
(#202296,#202297,#202298)),.UNSPECIFIED.,.F.,.F.,.F.)
B_SPLINE_SURFACE_WITH_KNOTS((4,2,4),(3,3),(0.,0.000257953807872846,0.000515907615745692),
(0.,1.),.UNSPECIFIED.)
GEOMETRIC_REPRESENTATION_ITEM()
RATIONAL_B_SPLINE_SURFACE(((1.,0.874619707139389,1.),(1.,0.874834349678646,
1.),(1.,0.854686104158268,1.),(1.,0.792476597914672,1.),(1.,0.75088785459547,
1.),(1.,0.705585838031423,1.)))
REPRESENTATION_ITEM('')
SURFACE()
);
#2762=(
BOUNDED_SURFACE()
B_SPLINE_SURFACE(3,2,((#202304,#202305,#202306),(#202307,#202308,#202309),
(#202310,#202311,#202312),(#202313,#202314,#202315)),.UNSPECIFIED.,.F.,
 .F.,.F.)
B_SPLINE_SURFACE_WITH_KNOTS((4,4),(3,3),(0.,0.000511815437699156),(0.,1.00105881331674),
 .UNSPECIFIED.)
GEOMETRIC_REPRESENTATION_ITEM()
RATIONAL_B_SPLINE_SURFACE(((1.,0.706796661946085,1.00062089519769),(1.,
0.707430821224981,1.00061955228511),(1.,0.708058545830442,1.00061822299877),
(1.,0.708394505252468,1.00061751156215)))
REPRESENTATION_ITEM('')
SURFACE()
);
#2763=(
BOUNDED_SURFACE()
B_SPLINE_SURFACE(3,2,((#202317,#202318,#202319),(#202320,#202321,#202322),
(#202323,#202324,#202325),(#202326,#202327,#202328),(#202329,#202330,#202331),
(#202332,#202333,#202334)),.UNSPECIFIED.,.F.,.F.,.F.)
B_SPLINE_SURFACE_WITH_KNOTS((4,2,4),(3,3),(2.71050543121376E-20,0.000256915317531266,
0.000513830635062532),(0.,1.),.UNSPECIFIED.)
GEOMETRIC_REPRESENTATION_ITEM()
RATIONAL_B_SPLINE_SURFACE(((1.,0.705585838031446,1.),(1.,0.750902433542212,
1.),(1.,0.792329530083219,1.),(1.,0.854288401593528,1.),(1.,0.874998031125645,
1.),(1.,0.874619707139392,1.)))
REPRESENTATION_ITEM('')
SURFACE()
);
#2764=(
BOUNDED_SURFACE()
B_SPLINE_SURFACE(3,2,((#202340,#202341,#202342),(#202343,#202344,#202345),
(#202346,#202347,#202348),(#202349,#202350,#202351),(#202352,#202353,#202354),
(#202355,#202356,#202357)),.UNSPECIFIED.,.F.,.F.,.F.)
B_SPLINE_SURFACE_WITH_KNOTS((4,2,4),(3,3),(-9.48676900924816E-18,0.000256592814262154,
0.000513185628524318),(0.,1.),.UNSPECIFIED.)
GEOMETRIC_REPRESENTATION_ITEM()
RATIONAL_B_SPLINE_SURFACE(((1.,0.708712527163665,1.),(1.,0.753780902613422,
1.),(1.,0.794538995769426,1.),(1.,0.855070770330873,1.),(1.,0.875018427445491,
1.),(1.,0.874619707139392,1.)))
REPRESENTATION_ITEM('')
SURFACE()
);
#2765=(
BOUNDED_SURFACE()
B_SPLINE_SURFACE(3,2,((#202359,#202360,#202361),(#202362,#202363,#202364),
(#202365,#202366,#202367),(#202368,#202369,#202370)),.UNSPECIFIED.,.F.,
 .F.,.F.)
B_SPLINE_SURFACE_WITH_KNOTS((4,4),(3,3),(0.,0.000511815072430408),(0.,1.0010559836591),
 .UNSPECIFIED.)
GEOMETRIC_REPRESENTATION_ITEM()
RATIONAL_B_SPLINE_SURFACE(((1.,0.70679749073362,1.00061923411718),(1.,0.706182062146524,
1.00062053388225),(1.,0.705584062768913,1.00062179683739),(1.,0.705266224770364,
1.00062246810085)))
REPRESENTATION_ITEM('')
SURFACE()
);
#2766=(
BOUNDED_SURFACE()
B_SPLINE_SURFACE(3,2,((#202376,#202377,#202378),(#202379,#202380,#202381),
(#202382,#202383,#202384),(#202385,#202386,#202387),(#202388,#202389,#202390),
(#202391,#202392,#202393)),.UNSPECIFIED.,.F.,.F.,.F.)
B_SPLINE_SURFACE_WITH_KNOTS((4,2,4),(3,3),(-9.40545384631175E-18,0.000257652232350876,
0.000515304464701762),(0.,1.),.UNSPECIFIED.)
GEOMETRIC_REPRESENTATION_ITEM()
RATIONAL_B_SPLINE_SURFACE(((1.,0.874619707139393,1.),(1.,0.874861180430243,
1.),(1.,0.855455725921459,1.),(1.,0.794699358954658,1.),(1.,0.753768977789092,
1.),(1.,0.70871252716366,1.)))
REPRESENTATION_ITEM('')
SURFACE()
);
#2767=(
BOUNDED_SURFACE()
B_SPLINE_SURFACE(3,2,((#202399,#202400,#202401),(#202402,#202403,#202404),
(#202405,#202406,#202407),(#202408,#202409,#202410)),.UNSPECIFIED.,.F.,
 .F.,.F.)
B_SPLINE_SURFACE_WITH_KNOTS((4,4),(3,3),(0.,0.000397394373651906),(0.,1.),
 .UNSPECIFIED.)
GEOMETRIC_REPRESENTATION_ITEM()
RATIONAL_B_SPLINE_SURFACE(((1.,0.707106781186548,1.),(1.,0.707752587915919,
1.),(1.,0.708377654540692,1.),(1.,0.708689770883306,1.)))
REPRESENTATION_ITEM('')
SURFACE()
);
#2768=(
BOUNDED_SURFACE()
B_SPLINE_SURFACE(3,2,((#202412,#202413,#202414),(#202415,#202416,#202417),
(#202418,#202419,#202420),(#202421,#202422,#202423)),.UNSPECIFIED.,.F.,
 .F.,.F.)
B_SPLINE_SURFACE_WITH_KNOTS((4,4),(3,3),(0.,0.000511815456479793),(0.,1.00105873159685),
 .UNSPECIFIED.)
GEOMETRIC_REPRESENTATION_ITEM()
RATIONAL_B_SPLINE_SURFACE(((1.,0.708394529057236,1.00061746385181),(1.,
0.708058564167794,1.00061817524509),(1.,0.707430835372963,1.00061950443771),
(1.,0.706796685881285,1.00062084722592)))
REPRESENTATION_ITEM('')
SURFACE()
);
#2769=(
BOUNDED_SURFACE()
B_SPLINE_SURFACE(3,2,((#202429,#202430,#202431),(#202432,#202433,#202434),
(#202435,#202436,#202437),(#202438,#202439,#202440)),.UNSPECIFIED.,.F.,
 .F.,.F.)
B_SPLINE_SURFACE_WITH_KNOTS((4,4),(3,3),(0.,0.000397394465448306),(0.,1.),
 .UNSPECIFIED.)
GEOMETRIC_REPRESENTATION_ITEM()
RATIONAL_B_SPLINE_SURFACE(((1.,0.705498956110745,1.),(1.,0.705821764811741,
1.),(1.,0.706461952521179,1.),(1.,0.707106781186536,1.)))
REPRESENTATION_ITEM('')
SURFACE()
);
#2770=(
BOUNDED_SURFACE()
B_SPLINE_SURFACE(3,2,((#202446,#202447,#202448),(#202449,#202450,#202451),
(#202452,#202453,#202454),(#202455,#202456,#202457)),.UNSPECIFIED.,.F.,
 .F.,.F.)
B_SPLINE_SURFACE_WITH_KNOTS((4,4),(3,3),(0.,0.00039739441082874),(0.,1.),
 .UNSPECIFIED.)
GEOMETRIC_REPRESENTATION_ITEM()
RATIONAL_B_SPLINE_SURFACE(((1.,0.708689770883326,1.),(1.,0.70837644003451,
1.),(1.,0.707750498698405,1.),(1.,0.707106781186548,1.)))
REPRESENTATION_ITEM('')
SURFACE()
);
#2771=(
BOUNDED_SURFACE()
B_SPLINE_SURFACE(3,2,((#202463,#202464,#202465),(#202466,#202467,#202468),
(#202469,#202470,#202471),(#202472,#202473,#202474)),.UNSPECIFIED.,.F.,
 .F.,.F.)
B_SPLINE_SURFACE_WITH_KNOTS((4,4),(3,3),(0.,0.000511815090126171),(0.,1.00105592270468),
 .UNSPECIFIED.)
GEOMETRIC_REPRESENTATION_ITEM()
RATIONAL_B_SPLINE_SURFACE(((1.,0.705266242716756,1.0006224321323),(1.,0.705584085908405,
1.00062176089661),(1.,0.706182089449784,1.00062049800558),(1.,0.706797508586757,
1.0006191983355)))
REPRESENTATION_ITEM('')
SURFACE()
);
#2772=(
BOUNDED_SURFACE()
B_SPLINE_SURFACE(3,2,((#202476,#202477,#202478),(#202479,#202480,#202481),
(#202482,#202483,#202484),(#202485,#202486,#202487)),.UNSPECIFIED.,.F.,
 .F.,.F.)
B_SPLINE_SURFACE_WITH_KNOTS((4,4),(3,3),(0.,0.000397394428086624),(0.,1.),
 .UNSPECIFIED.)
GEOMETRIC_REPRESENTATION_ITEM()
RATIONAL_B_SPLINE_SURFACE(((1.,0.707106781186548,1.),(1.,0.706459846759088,
1.),(1.,0.705820510737271,1.),(1.,0.705498956110742,1.)))
REPRESENTATION_ITEM('')
SURFACE()
);
#2773=(
BOUNDED_SURFACE()
B_SPLINE_SURFACE(3,2,((#202493,#202494,#202495),(#202496,#202497,#202498),
(#202499,#202500,#202501),(#202502,#202503,#202504),(#202505,#202506,#202507),
(#202508,#202509,#202510)),.UNSPECIFIED.,.F.,.F.,.F.)
B_SPLINE_SURFACE_WITH_KNOTS((4,2,4),(3,3),(0.,0.000257953807872849,0.000515907615745697),
(0.,1.),.UNSPECIFIED.)
GEOMETRIC_REPRESENTATION_ITEM()
RATIONAL_B_SPLINE_SURFACE(((1.,0.874619707139387,1.),(1.,0.874834349678404,
1.),(1.,0.854686104158593,1.),(1.,0.792476597914305,1.),(1.,0.750887854595777,
1.),(1.,0.705585838031401,1.)))
REPRESENTATION_ITEM('')
SURFACE()
);
#2774=(
BOUNDED_SURFACE()
B_SPLINE_SURFACE(3,2,((#202516,#202517,#202518),(#202519,#202520,#202521),
(#202522,#202523,#202524),(#202525,#202526,#202527)),.UNSPECIFIED.,.F.,
 .F.,.F.)
B_SPLINE_SURFACE_WITH_KNOTS((4,4),(3,3),(0.,0.000511815437699148),(0.,1.00105881331846),
 .UNSPECIFIED.)
GEOMETRIC_REPRESENTATION_ITEM()
RATIONAL_B_SPLINE_SURFACE(((1.,0.706796661945569,1.0006208951987),(1.,0.707430821224488,
1.00061955228611),(1.,0.708058545829957,1.00061822299977),(1.,0.708394505251976,
1.00061751156315)))
REPRESENTATION_ITEM('')
SURFACE()
);
#2775=(
BOUNDED_SURFACE()
B_SPLINE_SURFACE(3,2,((#202529,#202530,#202531),(#202532,#202533,#202534),
(#202535,#202536,#202537),(#202538,#202539,#202540),(#202541,#202542,#202543),
(#202544,#202545,#202546)),.UNSPECIFIED.,.F.,.F.,.F.)
B_SPLINE_SURFACE_WITH_KNOTS((4,2,4),(3,3),(0.,0.000256915317531259,0.000513830635062517),
(0.,1.),.UNSPECIFIED.)
GEOMETRIC_REPRESENTATION_ITEM()
RATIONAL_B_SPLINE_SURFACE(((1.,0.705585838031447,1.),(1.,0.750902433543016,
1.),(1.,0.792329530082168,1.),(1.,0.854288401594543,1.),(1.,0.874998031124862,
1.),(1.,0.874619707139394,1.)))
REPRESENTATION_ITEM('')
SURFACE()
);
#2776=(
BOUNDED_SURFACE()
B_SPLINE_SURFACE(3,2,((#202552,#202553,#202554),(#202555,#202556,#202557),
(#202558,#202559,#202560),(#202561,#202562,#202563),(#202564,#202565,#202566),
(#202567,#202568,#202569)),.UNSPECIFIED.,.F.,.F.,.F.)
B_SPLINE_SURFACE_WITH_KNOTS((4,2,4),(3,3),(0.,0.000256592814262157,0.000513185628524314),
(0.,1.),.UNSPECIFIED.)
GEOMETRIC_REPRESENTATION_ITEM()
RATIONAL_B_SPLINE_SURFACE(((1.,0.708712527163675,1.),(1.,0.753780902613242,
1.),(1.,0.794538995769671,1.),(1.,0.85507077033062,1.),(1.,0.875018427445703,
1.),(1.,0.874619707139387,1.)))
REPRESENTATION_ITEM('')
SURFACE()
);
#2777=(
BOUNDED_SURFACE()
B_SPLINE_SURFACE(3,2,((#202571,#202572,#202573),(#202574,#202575,#202576),
(#202577,#202578,#202579),(#202580,#202581,#202582)),.UNSPECIFIED.,.F.,
 .F.,.F.)
B_SPLINE_SURFACE_WITH_KNOTS((4,4),(3,3),(0.,0.000511815072430402),(0.,1.00105598365989),
 .UNSPECIFIED.)
GEOMETRIC_REPRESENTATION_ITEM()
RATIONAL_B_SPLINE_SURFACE(((1.,0.706797490733388,1.00061923411765),(1.,
0.70618206214629,1.00062053388271),(1.,0.70558406276869,1.00062179683786),
(1.,0.705266224770156,1.00062246810132)))
REPRESENTATION_ITEM('')
SURFACE()
);
#2778=(
BOUNDED_SURFACE()
B_SPLINE_SURFACE(3,2,((#202588,#202589,#202590),(#202591,#202592,#202593),
(#202594,#202595,#202596),(#202597,#202598,#202599),(#202600,#202601,#202602),
(#202603,#202604,#202605)),.UNSPECIFIED.,.F.,.F.,.F.)
B_SPLINE_SURFACE_WITH_KNOTS((4,2,4),(3,3),(0.,0.000257652232350882,0.000515304464701763),
(0.,1.),.UNSPECIFIED.)
GEOMETRIC_REPRESENTATION_ITEM()
RATIONAL_B_SPLINE_SURFACE(((1.,0.874619707139388,1.),(1.,0.874861180431117,
1.),(1.,0.855455725920339,1.),(1.,0.794699358955772,1.),(1.,0.753768977788269,
1.),(1.,0.70871252716366,1.)))
REPRESENTATION_ITEM('')
SURFACE()
);
#2779=(
BOUNDED_SURFACE()
B_SPLINE_SURFACE(3,2,((#202611,#202612,#202613),(#202614,#202615,#202616),
(#202617,#202618,#202619),(#202620,#202621,#202622)),.UNSPECIFIED.,.F.,
 .F.,.F.)
B_SPLINE_SURFACE_WITH_KNOTS((4,4),(3,3),(-1.47451495458029E-17,0.0003973943736519),
(0.,1.),.UNSPECIFIED.)
GEOMETRIC_REPRESENTATION_ITEM()
RATIONAL_B_SPLINE_SURFACE(((1.,0.707106781186548,1.),(1.,0.707752587915863,
1.),(1.,0.708377654540685,1.),(1.,0.708689770883324,1.)))
REPRESENTATION_ITEM('')
SURFACE()
);
#2780=(
BOUNDED_SURFACE()
B_SPLINE_SURFACE(3,2,((#202624,#202625,#202626),(#202627,#202628,#202629),
(#202630,#202631,#202632),(#202633,#202634,#202635)),.UNSPECIFIED.,.F.,
 .F.,.F.)
B_SPLINE_SURFACE_WITH_KNOTS((4,4),(3,3),(0.,0.000511815456479797),(0.,1.00105873159847),
 .UNSPECIFIED.)
GEOMETRIC_REPRESENTATION_ITEM()
RATIONAL_B_SPLINE_SURFACE(((1.,0.708394529056756,1.00061746385275),(1.,
0.708058564167281,1.00061817524604),(1.,0.707430835372509,1.00061950443866),
(1.,0.706796685880813,1.00062084722687)))
REPRESENTATION_ITEM('')
SURFACE()
);
#2781=(
BOUNDED_SURFACE()
B_SPLINE_SURFACE(3,2,((#202641,#202642,#202643),(#202644,#202645,#202646),
(#202647,#202648,#202649),(#202650,#202651,#202652)),.UNSPECIFIED.,.F.,
 .F.,.F.)
B_SPLINE_SURFACE_WITH_KNOTS((4,4),(3,3),(0.,0.000397394465448322),(0.,1.),
 .UNSPECIFIED.)
GEOMETRIC_REPRESENTATION_ITEM()
RATIONAL_B_SPLINE_SURFACE(((1.,0.705498956110752,1.),(1.,0.705821764811797,
1.),(1.,0.706461952521127,1.),(1.,0.707106781186548,1.)))
REPRESENTATION_ITEM('')
SURFACE()
);
#2782=(
BOUNDED_SURFACE()
B_SPLINE_SURFACE(3,2,((#202658,#202659,#202660),(#202661,#202662,#202663),
(#202664,#202665,#202666),(#202667,#202668,#202669)),.UNSPECIFIED.,.F.,
 .F.,.F.)
B_SPLINE_SURFACE_WITH_KNOTS((4,4),(3,3),(0.,0.000397394410828722),(0.,1.),
 .UNSPECIFIED.)
GEOMETRIC_REPRESENTATION_ITEM()
RATIONAL_B_SPLINE_SURFACE(((1.,0.708689770883299,1.),(1.,0.708376440034514,
1.),(1.,0.707750498698402,1.),(1.,0.707106781186535,1.)))
REPRESENTATION_ITEM('')
SURFACE()
);
#2783=(
BOUNDED_SURFACE()
B_SPLINE_SURFACE(3,2,((#202675,#202676,#202677),(#202678,#202679,#202680),
(#202681,#202682,#202683),(#202684,#202685,#202686)),.UNSPECIFIED.,.F.,
 .F.,.F.)
B_SPLINE_SURFACE_WITH_KNOTS((4,4),(3,3),(0.,0.000511815090126187),(0.,1.00105592270046),
 .UNSPECIFIED.)
GEOMETRIC_REPRESENTATION_ITEM()
RATIONAL_B_SPLINE_SURFACE(((1.,0.705266242718005,1.00062243212981),(1.,
0.705584085909643,1.00062176089413),(1.,0.706182089451007,1.0006204980031),
(1.,0.706797508587991,1.00061919833303)))
REPRESENTATION_ITEM('')
SURFACE()
);
#2784=(
BOUNDED_SURFACE()
B_SPLINE_SURFACE(3,2,((#202688,#202689,#202690),(#202691,#202692,#202693),
(#202694,#202695,#202696),(#202697,#202698,#202699)),.UNSPECIFIED.,.F.,
 .F.,.F.)
B_SPLINE_SURFACE_WITH_KNOTS((4,4),(3,3),(-1.47451495458029E-17,0.00039739442808661),
(0.,1.),.UNSPECIFIED.)
GEOMETRIC_REPRESENTATION_ITEM()
RATIONAL_B_SPLINE_SURFACE(((1.,0.707106781186549,1.),(1.,0.706459846759096,
1.),(1.,0.705820510737269,1.),(1.,0.705498956110752,1.)))
REPRESENTATION_ITEM('')
SURFACE()
);
#2785=(
BOUNDED_SURFACE()
B_SPLINE_SURFACE(3,2,((#202705,#202706,#202707),(#202708,#202709,#202710),
(#202711,#202712,#202713),(#202714,#202715,#202716),(#202717,#202718,#202719),
(#202720,#202721,#202722)),.UNSPECIFIED.,.F.,.F.,.F.)
B_SPLINE_SURFACE_WITH_KNOTS((4,2,4),(3,3),(0.,0.000257953807872851,0.000515907615745702),
(0.,1.),.UNSPECIFIED.)
GEOMETRIC_REPRESENTATION_ITEM()
RATIONAL_B_SPLINE_SURFACE(((1.,0.874619707139394,1.),(1.,0.874834349678836,
1.),(1.,0.85468610415798,1.),(1.,0.792476597914961,1.),(1.,0.750887854595252,
1.),(1.,0.705585838031447,1.)))
REPRESENTATION_ITEM('')
SURFACE()
);
#2786=(
BOUNDED_SURFACE()
B_SPLINE_SURFACE(3,2,((#202728,#202729,#202730),(#202731,#202732,#202733),
(#202734,#202735,#202736),(#202737,#202738,#202739)),.UNSPECIFIED.,.F.,
 .F.,.F.)
B_SPLINE_SURFACE_WITH_KNOTS((4,4),(3,3),(0.,0.000511815437699164),(0.,1.00105881331666),
 .UNSPECIFIED.)
GEOMETRIC_REPRESENTATION_ITEM()
RATIONAL_B_SPLINE_SURFACE(((1.,0.706796661946094,1.00062089519764),(1.,
0.707430821224998,1.00061955228506),(1.,0.708058545830475,1.00061822299872),
(1.,0.708394505252485,1.0006175115621)))
REPRESENTATION_ITEM('')
SURFACE()
);
#2787=(
BOUNDED_SURFACE()
B_SPLINE_SURFACE(3,2,((#202741,#202742,#202743),(#202744,#202745,#202746),
(#202747,#202748,#202749),(#202750,#202751,#202752),(#202753,#202754,#202755),
(#202756,#202757,#202758)),.UNSPECIFIED.,.F.,.F.,.F.)
B_SPLINE_SURFACE_WITH_KNOTS((4,2,4),(3,3),(0.,0.000256915317531265,0.000513830635062529),
(0.,1.),.UNSPECIFIED.)
GEOMETRIC_REPRESENTATION_ITEM()
RATIONAL_B_SPLINE_SURFACE(((1.,0.705585838031449,1.),(1.,0.750902433542386,
1.),(1.,0.792329530082973,1.),(1.,0.854288401593741,1.),(1.,0.874998031125484,
1.),(1.,0.874619707139406,1.)))
REPRESENTATION_ITEM('')
SURFACE()
);
#2788=(
BOUNDED_SURFACE()
B_SPLINE_SURFACE(3,2,((#202764,#202765,#202766),(#202767,#202768,#202769),
(#202770,#202771,#202772),(#202773,#202774,#202775),(#202776,#202777,#202778),
(#202779,#202780,#202781)),.UNSPECIFIED.,.F.,.F.,.F.)
B_SPLINE_SURFACE_WITH_KNOTS((4,2,4),(3,3),(-9.13440330319037E-18,0.000256592814262152,
0.000513185628524313),(0.,1.),.UNSPECIFIED.)
GEOMETRIC_REPRESENTATION_ITEM()
RATIONAL_B_SPLINE_SURFACE(((1.,0.708712527163635,1.),(1.,0.753780902613607,
1.),(1.,0.794538995769191,1.),(1.,0.855070770331096,1.),(1.,0.875018427445334,
1.),(1.,0.874619707139393,1.)))
REPRESENTATION_ITEM('')
SURFACE()
);
#2789=(
BOUNDED_SURFACE()
B_SPLINE_SURFACE(3,2,((#202783,#202784,#202785),(#202786,#202787,#202788),
(#202789,#202790,#202791),(#202792,#202793,#202794)),.UNSPECIFIED.,.F.,
 .F.,.F.)
B_SPLINE_SURFACE_WITH_KNOTS((4,4),(3,3),(-2.71050543121376E-20,0.000511815072430406),
(0.,1.00105598365961),.UNSPECIFIED.)
GEOMETRIC_REPRESENTATION_ITEM()
RATIONAL_B_SPLINE_SURFACE(((1.,0.706797490733471,1.00061923411748),(1.,
0.706182062146368,1.00062053388255),(1.,0.705584062768763,1.00062179683769),
(1.,0.705266224770216,1.00062246810115)))
REPRESENTATION_ITEM('')
SURFACE()
);
#2790=(
BOUNDED_SURFACE()
B_SPLINE_SURFACE(3,2,((#202800,#202801,#202802),(#202803,#202804,#202805),
(#202806,#202807,#202808),(#202809,#202810,#202811),(#202812,#202813,#202814),
(#202815,#202816,#202817)),.UNSPECIFIED.,.F.,.F.,.F.)
B_SPLINE_SURFACE_WITH_KNOTS((4,2,4),(3,3),(-5.02798757490153E-18,0.000257652232350882,
0.00051530446470177),(0.,1.),.UNSPECIFIED.)
GEOMETRIC_REPRESENTATION_ITEM()
RATIONAL_B_SPLINE_SURFACE(((1.,0.874619707139381,1.),(1.,0.87486118043123,
1.),(1.,0.855455725920156,1.),(1.,0.794699358955984,1.),(1.,0.753768977788076,
1.),(1.,0.708712527163675,1.)))
REPRESENTATION_ITEM('')
SURFACE()
);
#2791=(
BOUNDED_SURFACE()
B_SPLINE_SURFACE(3,2,((#202823,#202824,#202825),(#202826,#202827,#202828),
(#202829,#202830,#202831),(#202832,#202833,#202834)),.UNSPECIFIED.,.F.,
 .F.,.F.)
B_SPLINE_SURFACE_WITH_KNOTS((4,4),(3,3),(0.,0.000397394373651916),(0.,1.),
 .UNSPECIFIED.)
GEOMETRIC_REPRESENTATION_ITEM()
RATIONAL_B_SPLINE_SURFACE(((1.,0.707106781186535,1.),(1.,0.707752587915909,
1.),(1.,0.708377654540687,1.),(1.,0.708689770883326,1.)))
REPRESENTATION_ITEM('')
SURFACE()
);
#2792=(
BOUNDED_SURFACE()
B_SPLINE_SURFACE(3,2,((#202836,#202837,#202838),(#202839,#202840,#202841),
(#202842,#202843,#202844),(#202845,#202846,#202847)),.UNSPECIFIED.,.F.,
 .F.,.F.)
B_SPLINE_SURFACE_WITH_KNOTS((4,4),(3,3),(0.,0.00051181545647979),(0.,1.0010587315986),
 .UNSPECIFIED.)
GEOMETRIC_REPRESENTATION_ITEM()
RATIONAL_B_SPLINE_SURFACE(((1.,0.708394529056717,1.00061746385283),(1.,
0.70805856416728,1.00061817524611),(1.,0.70743083537246,1.00061950443873),
(1.,0.706796685880774,1.00062084722695)))
REPRESENTATION_ITEM('')
SURFACE()
);
#2793=(
BOUNDED_SURFACE()
B_SPLINE_SURFACE(3,2,((#202853,#202854,#202855),(#202856,#202857,#202858),
(#202859,#202860,#202861),(#202862,#202863,#202864)),.UNSPECIFIED.,.F.,
 .F.,.F.)
B_SPLINE_SURFACE_WITH_KNOTS((4,4),(3,3),(0.,0.000397394465448294),(0.,1.),
 .UNSPECIFIED.)
GEOMETRIC_REPRESENTATION_ITEM()
RATIONAL_B_SPLINE_SURFACE(((1.,0.705498956110742,1.),(1.,0.705821764811805,
1.),(1.,0.706461952521124,1.),(1.,0.70710678118656,1.)))
REPRESENTATION_ITEM('')
SURFACE()
);
#2794=(
BOUNDED_SURFACE()
B_SPLINE_SURFACE(3,2,((#202870,#202871,#202872),(#202873,#202874,#202875),
(#202876,#202877,#202878),(#202879,#202880,#202881)),.UNSPECIFIED.,.F.,
 .F.,.F.)
B_SPLINE_SURFACE_WITH_KNOTS((4,4),(3,3),(0.,0.00039739441082874),(0.,1.),
 .UNSPECIFIED.)
GEOMETRIC_REPRESENTATION_ITEM()
RATIONAL_B_SPLINE_SURFACE(((1.,0.708689770883332,1.),(1.,0.708376440034517,
1.),(1.,0.70775049869838,1.),(1.,0.707106781186548,1.)))
REPRESENTATION_ITEM('')
SURFACE()
);
#2795=(
BOUNDED_SURFACE()
B_SPLINE_SURFACE(3,2,((#202887,#202888,#202889),(#202890,#202891,#202892),
(#202893,#202894,#202895),(#202896,#202897,#202898)),.UNSPECIFIED.,.F.,
 .F.,.F.)
B_SPLINE_SURFACE_WITH_KNOTS((4,4),(3,3),(0.,0.000511815090126175),(0.,1.00105592270174),
 .UNSPECIFIED.)
GEOMETRIC_REPRESENTATION_ITEM()
RATIONAL_B_SPLINE_SURFACE(((1.,0.705266242717628,1.00062243213056),(1.,
0.705584085909269,1.00062176089488),(1.,0.706182089450612,1.00062049800385),
(1.,0.706797508587618,1.00061919833378)))
REPRESENTATION_ITEM('')
SURFACE()
);
#2796=(
BOUNDED_SURFACE()
B_SPLINE_SURFACE(3,2,((#202900,#202901,#202902),(#202903,#202904,#202905),
(#202906,#202907,#202908),(#202909,#202910,#202911)),.UNSPECIFIED.,.F.,
 .F.,.F.)
B_SPLINE_SURFACE_WITH_KNOTS((4,4),(3,3),(0.,0.000397394428086641),(0.,1.),
 .UNSPECIFIED.)
GEOMETRIC_REPRESENTATION_ITEM()
RATIONAL_B_SPLINE_SURFACE(((1.,0.707106781186532,1.),(1.,0.706459846759111,
1.),(1.,0.705820510737279,1.),(1.,0.705498956110745,1.)))
REPRESENTATION_ITEM('')
SURFACE()
);
#2797=(
BOUNDED_SURFACE()
B_SPLINE_SURFACE(3,2,((#202917,#202918,#202919),(#202920,#202921,#202922),
(#202923,#202924,#202925),(#202926,#202927,#202928),(#202929,#202930,#202931),
(#202932,#202933,#202934)),.UNSPECIFIED.,.F.,.F.,.F.)
B_SPLINE_SURFACE_WITH_KNOTS((4,2,4),(3,3),(0.,0.000257953807872849,0.000515907615745698),
(0.,1.),.UNSPECIFIED.)
GEOMETRIC_REPRESENTATION_ITEM()
RATIONAL_B_SPLINE_SURFACE(((1.,0.874619707139397,1.),(1.,0.874834349679158,
1.),(1.,0.854686104157565,1.),(1.,0.792476597915372,1.),(1.,0.750887854594947,
1.),(1.,0.705585838031446,1.)))
REPRESENTATION_ITEM('')
SURFACE()
);
#2798=(
BOUNDED_SURFACE()
B_SPLINE_SURFACE(3,2,((#202940,#202941,#202942),(#202943,#202944,#202945),
(#202946,#202947,#202948),(#202949,#202950,#202951)),.UNSPECIFIED.,.F.,
 .F.,.F.)
B_SPLINE_SURFACE_WITH_KNOTS((4,4),(3,3),(0.,0.000511815437699156),(0.,1.00105881331736),
 .UNSPECIFIED.)
GEOMETRIC_REPRESENTATION_ITEM()
RATIONAL_B_SPLINE_SURFACE(((1.,0.706796661945893,1.00062089519805),(1.,
0.707430821224857,1.00061955228547),(1.,0.708058545830205,1.00061822299913),
(1.,0.708394505252324,1.00061751156251)))
REPRESENTATION_ITEM('')
SURFACE()
);
#2799=(
BOUNDED_SURFACE()
B_SPLINE_SURFACE(3,2,((#202953,#202954,#202955),(#202956,#202957,#202958),
(#202959,#202960,#202961),(#202962,#202963,#202964),(#202965,#202966,#202967),
(#202968,#202969,#202970)),.UNSPECIFIED.,.F.,.F.,.F.)
B_SPLINE_SURFACE_WITH_KNOTS((4,2,4),(3,3),(-2.71050543121376E-20,0.000256915317531263,
0.000513830635062526),(0.,1.),.UNSPECIFIED.)
GEOMETRIC_REPRESENTATION_ITEM()
RATIONAL_B_SPLINE_SURFACE(((1.,0.705585838031448,1.),(1.,0.750902433542692,
1.),(1.,0.792329530082588,1.),(1.,0.854288401594132,1.),(1.,0.874998031125192,
1.),(1.,0.874619707139397,1.)))
REPRESENTATION_ITEM('')
SURFACE()
);
#2800=(
BOUNDED_SURFACE()
B_SPLINE_SURFACE(3,2,((#202976,#202977,#202978),(#202979,#202980,#202981),
(#202982,#202983,#202984),(#202985,#202986,#202987),(#202988,#202989,#202990),
(#202991,#202992,#202993)),.UNSPECIFIED.,.F.,.F.,.F.)
B_SPLINE_SURFACE_WITH_KNOTS((4,2,4),(3,3),(0.,0.000256592814262158,0.000513185628524316),
(0.,1.),.UNSPECIFIED.)
GEOMETRIC_REPRESENTATION_ITEM()
RATIONAL_B_SPLINE_SURFACE(((1.,0.708712527163647,1.),(1.,0.753780902613447,
1.),(1.,0.794538995769415,1.),(1.,0.855070770330899,1.),(1.,0.875018427445479,
1.),(1.,0.874619707139393,1.)))
REPRESENTATION_ITEM('')
SURFACE()
);
#2801=(
BOUNDED_SURFACE()
B_SPLINE_SURFACE(3,2,((#202995,#202996,#202997),(#202998,#202999,#203000),
(#203001,#203002,#203003),(#203004,#203005,#203006)),.UNSPECIFIED.,.F.,
 .F.,.F.)
B_SPLINE_SURFACE_WITH_KNOTS((4,4),(3,3),(0.,0.000511815072430398),(0.,1.00105598365643),
 .UNSPECIFIED.)
GEOMETRIC_REPRESENTATION_ITEM()
RATIONAL_B_SPLINE_SURFACE(((1.,0.70679749073439,1.00061923411562),(1.,0.706182062147315,
1.00062053388068),(1.,0.705584062769728,1.00062179683581),(1.,0.705266224771143,
1.00062246809928)))
REPRESENTATION_ITEM('')
SURFACE()
);
#2802=(
BOUNDED_SURFACE()
B_SPLINE_SURFACE(3,2,((#203012,#203013,#203014),(#203015,#203016,#203017),
(#203018,#203019,#203020),(#203021,#203022,#203023),(#203024,#203025,#203026),
(#203027,#203028,#203029)),.UNSPECIFIED.,.F.,.F.,.F.)
B_SPLINE_SURFACE_WITH_KNOTS((4,2,4),(3,3),(0.,0.000257652232350883,0.000515304464701767),
(0.,1.),.UNSPECIFIED.)
GEOMETRIC_REPRESENTATION_ITEM()
RATIONAL_B_SPLINE_SURFACE(((1.,0.874619707139392,1.),(1.,0.874861180430632,
1.),(1.,0.855455725920956,1.),(1.,0.794699358955172,1.),(1.,0.753768977788696,
1.),(1.,0.70871252716365,1.)))
REPRESENTATION_ITEM('')
SURFACE()
);
#2803=(
BOUNDED_SURFACE()
B_SPLINE_SURFACE(3,2,((#203035,#203036,#203037),(#203038,#203039,#203040),
(#203041,#203042,#203043),(#203044,#203045,#203046)),.UNSPECIFIED.,.F.,
 .F.,.F.)
B_SPLINE_SURFACE_WITH_KNOTS((4,4),(3,3),(0.,0.000397394373651906),(0.,1.),
 .UNSPECIFIED.)
GEOMETRIC_REPRESENTATION_ITEM()
RATIONAL_B_SPLINE_SURFACE(((1.,0.707106781186548,1.),(1.,0.707752587915907,
1.),(1.,0.70837765454067,1.),(1.,0.708689770883331,1.)))
REPRESENTATION_ITEM('')
SURFACE()
);
#2804=(
BOUNDED_SURFACE()
B_SPLINE_SURFACE(3,2,((#203048,#203049,#203050),(#203051,#203052,#203053),
(#203054,#203055,#203056),(#203057,#203058,#203059)),.UNSPECIFIED.,.F.,
 .F.,.F.)
B_SPLINE_SURFACE_WITH_KNOTS((4,4),(3,3),(-6.42389787197661E-18,0.000511815456479789),
(0.,1.00105873159726),.UNSPECIFIED.)
GEOMETRIC_REPRESENTATION_ITEM()
RATIONAL_B_SPLINE_SURFACE(((1.,0.708394529057106,1.00061746385204),(1.,
0.70805856416768,1.00061817524533),(1.,0.707430835372831,1.00061950443795),
(1.,0.706796685881154,1.00062084722616)))
REPRESENTATION_ITEM('')
SURFACE()
);
#2805=(
BOUNDED_SURFACE()
B_SPLINE_SURFACE(3,2,((#203065,#203066,#203067),(#203068,#203069,#203070),
(#203071,#203072,#203073),(#203074,#203075,#203076)),.UNSPECIFIED.,.F.,
 .F.,.F.)
B_SPLINE_SURFACE_WITH_KNOTS((4,4),(3,3),(0.,0.000397394465448304),(0.,1.),
 .UNSPECIFIED.)
GEOMETRIC_REPRESENTATION_ITEM()
RATIONAL_B_SPLINE_SURFACE(((1.,0.705498956110752,1.),(1.,0.705821764811813,
1.),(1.,0.706461952521096,1.),(1.,0.707106781186559,1.)))
REPRESENTATION_ITEM('')
SURFACE()
);
#2806=(
BOUNDED_SURFACE()
B_SPLINE_SURFACE(3,2,((#203082,#203083,#203084),(#203085,#203086,#203087),
(#203088,#203089,#203090),(#203091,#203092,#203093)),.UNSPECIFIED.,.F.,
 .F.,.F.)
B_SPLINE_SURFACE_WITH_KNOTS((4,4),(3,3),(0.,0.000397394410828728),(0.,1.),
 .UNSPECIFIED.)
GEOMETRIC_REPRESENTATION_ITEM()
RATIONAL_B_SPLINE_SURFACE(((1.,0.708689770883344,1.),(1.,0.708376440034511,
1.),(1.,0.707750498698398,1.),(1.,0.707106781186548,1.)))
REPRESENTATION_ITEM('')
SURFACE()
);
#2807=(
BOUNDED_SURFACE()
B_SPLINE_SURFACE(3,2,((#203099,#203100,#203101),(#203102,#203103,#203104),
(#203105,#203106,#203107),(#203108,#203109,#203110)),.UNSPECIFIED.,.F.,
 .F.,.F.)
B_SPLINE_SURFACE_WITH_KNOTS((4,4),(3,3),(0.,0.000511815090126177),(0.,1.00105592270118),
 .UNSPECIFIED.)
GEOMETRIC_REPRESENTATION_ITEM()
RATIONAL_B_SPLINE_SURFACE(((1.,0.705266242717771,1.00062243213024),(1.,
0.705584085909434,1.00062176089455),(1.,0.706182089450805,1.00062049800353),
(1.,0.70679750858778,1.00061919833345)))
REPRESENTATION_ITEM('')
SURFACE()
);
#2808=(
BOUNDED_SURFACE()
B_SPLINE_SURFACE(3,2,((#203112,#203113,#203114),(#203115,#203116,#203117),
(#203118,#203119,#203120),(#203121,#203122,#203123)),.UNSPECIFIED.,.F.,
 .F.,.F.)
B_SPLINE_SURFACE_WITH_KNOTS((4,4),(3,3),(0.,0.000397394428086627),(0.,1.),
 .UNSPECIFIED.)
GEOMETRIC_REPRESENTATION_ITEM()
RATIONAL_B_SPLINE_SURFACE(((1.,0.707106781186549,1.),(1.,0.706459846759132,
1.),(1.,0.705820510737241,1.),(1.,0.705498956110748,1.)))
REPRESENTATION_ITEM('')
SURFACE()
);
#2809=(
BOUNDED_SURFACE()
B_SPLINE_SURFACE(3,2,((#203129,#203130,#203131),(#203132,#203133,#203134),
(#203135,#203136,#203137),(#203138,#203139,#203140),(#203141,#203142,#203143),
(#203144,#203145,#203146)),.UNSPECIFIED.,.F.,.F.,.F.)
B_SPLINE_SURFACE_WITH_KNOTS((4,2,4),(3,3),(0.,0.000257953807872846,0.000515907615745692),
(0.,1.),.UNSPECIFIED.)
GEOMETRIC_REPRESENTATION_ITEM()
RATIONAL_B_SPLINE_SURFACE(((1.,0.874619707139383,1.),(1.,0.874834349679598,
1.),(1.,0.854686104157003,1.),(1.,0.792476597915936,1.),(1.,0.750887854594542,
1.),(1.,0.705585838031438,1.)))
REPRESENTATION_ITEM('')
SURFACE()
);
#2810=(
BOUNDED_SURFACE()
B_SPLINE_SURFACE(3,2,((#203152,#203153,#203154),(#203155,#203156,#203157),
(#203158,#203159,#203160),(#203161,#203162,#203163)),.UNSPECIFIED.,.F.,
 .F.,.F.)
B_SPLINE_SURFACE_WITH_KNOTS((4,4),(3,3),(0.,0.000511815437699146),(0.,1.00105881331538),
 .UNSPECIFIED.)
GEOMETRIC_REPRESENTATION_ITEM()
RATIONAL_B_SPLINE_SURFACE(((1.,0.706796661946483,1.00062089519689),(1.,
0.70743082122537,1.00061955228431),(1.,0.708058545830867,1.00061822299797),
(1.,0.708394505252865,1.00061751156135)))
REPRESENTATION_ITEM('')
SURFACE()
);
#2811=(
BOUNDED_SURFACE()
B_SPLINE_SURFACE(3,2,((#203165,#203166,#203167),(#203168,#203169,#203170),
(#203171,#203172,#203173),(#203174,#203175,#203176),(#203177,#203178,#203179),
(#203180,#203181,#203182)),.UNSPECIFIED.,.F.,.F.,.F.)
B_SPLINE_SURFACE_WITH_KNOTS((4,2,4),(3,3),(0.,0.000256915317531269,0.000513830635062538),
(0.,1.),.UNSPECIFIED.)
GEOMETRIC_REPRESENTATION_ITEM()
RATIONAL_B_SPLINE_SURFACE(((1.,0.705585838031449,1.),(1.,0.75090243354275,
1.),(1.,0.792329530082535,1.),(1.,0.854288401594234,1.),(1.,0.874998031125134,
1.),(1.,0.874619707139408,1.)))
REPRESENTATION_ITEM('')
SURFACE()
);
#2812=(
BOUNDED_SURFACE()
B_SPLINE_SURFACE(3,2,((#203188,#203189,#203190),(#203191,#203192,#203193),
(#203194,#203195,#203196),(#203197,#203198,#203199),(#203200,#203201,#203202),
(#203203,#203204,#203205)),.UNSPECIFIED.,.F.,.F.,.F.)
B_SPLINE_SURFACE_WITH_KNOTS((4,2,4),(3,3),(-9.7307144980574E-18,0.000256592814262153,
0.000513185628524316),(0.,1.),.UNSPECIFIED.)
GEOMETRIC_REPRESENTATION_ITEM()
RATIONAL_B_SPLINE_SURFACE(((1.,0.708712527163667,1.),(1.,0.7537809026138,
1.),(1.,0.79453899576896,1.),(1.,0.855070770331341,1.),(1.,0.875018427445144,
1.),(1.,0.874619707139388,1.)))
REPRESENTATION_ITEM('')
SURFACE()
);
#2813=(
BOUNDED_SURFACE()
B_SPLINE_SURFACE(3,2,((#203207,#203208,#203209),(#203210,#203211,#203212),
(#203213,#203214,#203215),(#203216,#203217,#203218)),.UNSPECIFIED.,.F.,
 .F.,.F.)
B_SPLINE_SURFACE_WITH_KNOTS((4,4),(3,3),(0.,0.000511815072430414),(0.,1.00105598365751),
 .UNSPECIFIED.)
GEOMETRIC_REPRESENTATION_ITEM()
RATIONAL_B_SPLINE_SURFACE(((1.,0.706797490734085,1.00061923411625),(1.,
0.70618206214702,1.00062053388131),(1.,0.705584062769344,1.00062179683645),
(1.,0.70526622477087,1.00062246809992)))
REPRESENTATION_ITEM('')
SURFACE()
);
#2814=(
BOUNDED_SURFACE()
B_SPLINE_SURFACE(3,2,((#203224,#203225,#203226),(#203227,#203228,#203229),
(#203230,#203231,#203232),(#203233,#203234,#203235),(#203236,#203237,#203238),
(#203239,#203240,#203241)),.UNSPECIFIED.,.F.,.F.,.F.)
B_SPLINE_SURFACE_WITH_KNOTS((4,2,4),(3,3),(0.,0.00025765223235089,0.00051530446470178),
(0.,1.),.UNSPECIFIED.)
GEOMETRIC_REPRESENTATION_ITEM()
RATIONAL_B_SPLINE_SURFACE(((1.,0.874619707139373,1.),(1.,0.874861180430774,
1.),(1.,0.855455725920732,1.),(1.,0.79469935895536,1.),(1.,0.75376897778856,
1.),(1.,0.708712527163633,1.)))
REPRESENTATION_ITEM('')
SURFACE()
);
#2815=(
BOUNDED_SURFACE()
B_SPLINE_SURFACE(3,2,((#203247,#203248,#203249),(#203250,#203251,#203252),
(#203253,#203254,#203255),(#203256,#203257,#203258)),.UNSPECIFIED.,.F.,
 .F.,.F.)
B_SPLINE_SURFACE_WITH_KNOTS((4,4),(3,3),(0.,0.000397394373651923),(0.,1.),
 .UNSPECIFIED.)
GEOMETRIC_REPRESENTATION_ITEM()
RATIONAL_B_SPLINE_SURFACE(((1.,0.707106781186548,1.),(1.,0.707752587915923,
1.),(1.,0.708377654540652,1.),(1.,0.708689770883338,1.)))
REPRESENTATION_ITEM('')
SURFACE()
);
#2816=(
BOUNDED_SURFACE()
B_SPLINE_SURFACE(3,2,((#203260,#203261,#203262),(#203263,#203264,#203265),
(#203266,#203267,#203268),(#203269,#203270,#203271)),.UNSPECIFIED.,.F.,
 .F.,.F.)
B_SPLINE_SURFACE_WITH_KNOTS((4,4),(3,3),(-6.42389787197661E-18,0.00051181545647979),
(0.,1.00105873159723),.UNSPECIFIED.)
GEOMETRIC_REPRESENTATION_ITEM()
RATIONAL_B_SPLINE_SURFACE(((1.,0.708394529057117,1.00061746385203),(1.,
0.708058564167685,1.00061817524531),(1.,0.707430835372828,1.00061950443793),
(1.,0.706796685881165,1.00062084722614)))
REPRESENTATION_ITEM('')
SURFACE()
);
#2817=(
BOUNDED_SURFACE()
B_SPLINE_SURFACE(3,2,((#203277,#203278,#203279),(#203280,#203281,#203282),
(#203283,#203284,#203285),(#203286,#203287,#203288)),.UNSPECIFIED.,.F.,
 .F.,.F.)
B_SPLINE_SURFACE_WITH_KNOTS((4,4),(3,3),(-1.57209315010398E-17,0.000397394465448301),
(0.,1.),.UNSPECIFIED.)
GEOMETRIC_REPRESENTATION_ITEM()
RATIONAL_B_SPLINE_SURFACE(((1.,0.705498956110757,1.),(1.,0.705821764811813,
1.),(1.,0.706461952521126,1.),(1.,0.707106781186557,1.)))
REPRESENTATION_ITEM('')
SURFACE()
);
#2818=(
BOUNDED_SURFACE()
B_SPLINE_SURFACE(3,2,((#203294,#203295,#203296),(#203297,#203298,#203299),
(#203300,#203301,#203302),(#203303,#203304,#203305)),.UNSPECIFIED.,.F.,
 .F.,.F.)
B_SPLINE_SURFACE_WITH_KNOTS((4,4),(3,3),(0.,0.000397394410828746),(0.,1.),
 .UNSPECIFIED.)
GEOMETRIC_REPRESENTATION_ITEM()
RATIONAL_B_SPLINE_SURFACE(((1.,0.708689770883336,1.),(1.,0.708376440034495,
1.),(1.,0.707750498698418,1.),(1.,0.707106781186547,1.)))
REPRESENTATION_ITEM('')
SURFACE()
);
#2819=(
BOUNDED_SURFACE()
B_SPLINE_SURFACE(3,2,((#203311,#203312,#203313),(#203314,#203315,#203316),
(#203317,#203318,#203319),(#203320,#203321,#203322)),.UNSPECIFIED.,.F.,
 .F.,.F.)
B_SPLINE_SURFACE_WITH_KNOTS((4,4),(3,3),(0.,0.000511815090126181),(0.,1.0010559227012),
 .UNSPECIFIED.)
GEOMETRIC_REPRESENTATION_ITEM()
RATIONAL_B_SPLINE_SURFACE(((1.,0.705266242717788,1.00062243213025),(1.,
0.705584085909427,1.00062176089456),(1.,0.706182089450776,1.00062049800353),
(1.,0.706797508587784,1.00061919833346)))
REPRESENTATION_ITEM('')
SURFACE()
);
#2820=(
BOUNDED_SURFACE()
B_SPLINE_SURFACE(3,2,((#203324,#203325,#203326),(#203327,#203328,#203329),
(#203330,#203331,#203332),(#203333,#203334,#203335)),.UNSPECIFIED.,.F.,
 .F.,.F.)
B_SPLINE_SURFACE_WITH_KNOTS((4,4),(3,3),(0.,0.00039739442808663),(0.,1.),
 .UNSPECIFIED.)
GEOMETRIC_REPRESENTATION_ITEM()
RATIONAL_B_SPLINE_SURFACE(((1.,0.707106781186539,1.),(1.,0.706459846759109,
1.),(1.,0.705820510737253,1.),(1.,0.705498956110755,1.)))
REPRESENTATION_ITEM('')
SURFACE()
);
#2821=(
BOUNDED_SURFACE()
B_SPLINE_SURFACE(3,2,((#203341,#203342,#203343),(#203344,#203345,#203346),
(#203347,#203348,#203349),(#203350,#203351,#203352),(#203353,#203354,#203355),
(#203356,#203357,#203358)),.UNSPECIFIED.,.F.,.F.,.F.)
B_SPLINE_SURFACE_WITH_KNOTS((4,2,4),(3,3),(0.,0.000257953807872851,0.000515907615745702),
(0.,1.),.UNSPECIFIED.)
GEOMETRIC_REPRESENTATION_ITEM()
RATIONAL_B_SPLINE_SURFACE(((1.,0.874619707139387,1.),(1.,0.874834349679411,
1.),(1.,0.854686104157238,1.),(1.,0.792476597915689,1.),(1.,0.750887854594714,
1.),(1.,0.705585838031445,1.)))
REPRESENTATION_ITEM('')
SURFACE()
);
#2822=(
BOUNDED_SURFACE()
B_SPLINE_SURFACE(3,2,((#203364,#203365,#203366),(#203367,#203368,#203369),
(#203370,#203371,#203372),(#203373,#203374,#203375)),.UNSPECIFIED.,.F.,
 .F.,.F.)
B_SPLINE_SURFACE_WITH_KNOTS((4,4),(3,3),(0.,0.000511815437699153),(0.,1.00105881331596),
 .UNSPECIFIED.)
GEOMETRIC_REPRESENTATION_ITEM()
RATIONAL_B_SPLINE_SURFACE(((1.,0.706796661946323,1.00062089519723),(1.,
0.707430821225177,1.00061955228465),(1.,0.708058545830703,1.00061822299831),
(1.,0.708394505252707,1.00061751156169)))
REPRESENTATION_ITEM('')
SURFACE()
);
#2823=(
BOUNDED_SURFACE()
B_SPLINE_SURFACE(3,2,((#203377,#203378,#203379),(#203380,#203381,#203382),
(#203383,#203384,#203385),(#203386,#203387,#203388),(#203389,#203390,#203391),
(#203392,#203393,#203394)),.UNSPECIFIED.,.F.,.F.,.F.)
B_SPLINE_SURFACE_WITH_KNOTS((4,2,4),(3,3),(0.,0.000256915317531267,0.000513830635062533),
(0.,1.),.UNSPECIFIED.)
GEOMETRIC_REPRESENTATION_ITEM()
RATIONAL_B_SPLINE_SURFACE(((1.,0.705585838031441,1.),(1.,0.750902433542965,
1.),(1.,0.792329530082225,1.),(1.,0.854288401594516,1.),(1.,0.874998031124923,
1.),(1.,0.874619707139399,1.)))
REPRESENTATION_ITEM('')
SURFACE()
);
#2824=(
BOUNDED_SURFACE()
B_SPLINE_SURFACE(3,2,((#203400,#203401,#203402),(#203403,#203404,#203405),
(#203406,#203407,#203408),(#203409,#203410,#203411),(#203412,#203413,#203414),
(#203415,#203416,#203417)),.UNSPECIFIED.,.F.,.F.,.F.)
B_SPLINE_SURFACE_WITH_KNOTS((4,2,4),(3,3),(-9.86623976961809E-18,0.000256592814262151,
0.000513185628524312),(0.,1.),.UNSPECIFIED.)
GEOMETRIC_REPRESENTATION_ITEM()
RATIONAL_B_SPLINE_SURFACE(((1.,0.708712527163664,1.),(1.,0.753780902613921,
1.),(1.,0.794538995768751,1.),(1.,0.855070770331543,1.),(1.,0.875018427444988,
1.),(1.,0.874619707139397,1.)))
REPRESENTATION_ITEM('')
SURFACE()
);
#2825=(
BOUNDED_SURFACE()
B_SPLINE_SURFACE(3,2,((#203419,#203420,#203421),(#203422,#203423,#203424),
(#203425,#203426,#203427),(#203428,#203429,#203430)),.UNSPECIFIED.,.F.,
 .F.,.F.)
B_SPLINE_SURFACE_WITH_KNOTS((4,4),(3,3),(0.,0.000511815072430393),(0.,1.00105598365616),
 .UNSPECIFIED.)
GEOMETRIC_REPRESENTATION_ITEM()
RATIONAL_B_SPLINE_SURFACE(((1.,0.706797490734472,1.00061923411546),(1.,
0.706182062147432,1.00062053388052),(1.,0.70558406276972,1.00062179683566),
(1.,0.705266224771268,1.00062246809912)))
REPRESENTATION_ITEM('')
SURFACE()
);
#2826=(
BOUNDED_SURFACE()
B_SPLINE_SURFACE(3,2,((#203436,#203437,#203438),(#203439,#203440,#203441),
(#203442,#203443,#203444),(#203445,#203446,#203447),(#203448,#203449,#203450),
(#203451,#203452,#203453)),.UNSPECIFIED.,.F.,.F.,.F.)
B_SPLINE_SURFACE_WITH_KNOTS((4,2,4),(3,3),(0.,0.000257652232350879,0.000515304464701758),
(0.,1.),.UNSPECIFIED.)
GEOMETRIC_REPRESENTATION_ITEM()
RATIONAL_B_SPLINE_SURFACE(((1.,0.874619707139378,1.),(1.,0.87486118043099,
1.),(1.,0.855455725920465,1.),(1.,0.794699358955661,1.),(1.,0.753768977788322,
1.),(1.,0.70871252716365,1.)))
REPRESENTATION_ITEM('')
SURFACE()
);
#2827=(
BOUNDED_SURFACE()
B_SPLINE_SURFACE(3,2,((#203459,#203460,#203461),(#203462,#203463,#203464),
(#203465,#203466,#203467),(#203468,#203469,#203470)),.UNSPECIFIED.,.F.,
 .F.,.F.)
B_SPLINE_SURFACE_WITH_KNOTS((4,4),(3,3),(0.,0.000397394373651913),(0.,1.),
 .UNSPECIFIED.)
GEOMETRIC_REPRESENTATION_ITEM()
RATIONAL_B_SPLINE_SURFACE(((1.,0.70710678118654,1.),(1.,0.707752587915909,
1.),(1.,0.708377654540683,1.),(1.,0.708689770883316,1.)))
REPRESENTATION_ITEM('')
SURFACE()
);
#2828=(
BOUNDED_SURFACE()
B_SPLINE_SURFACE(3,2,((#203472,#203473,#203474),(#203475,#203476,#203477),
(#203478,#203479,#203480),(#203481,#203482,#203483)),.UNSPECIFIED.,.F.,
 .F.,.F.)
B_SPLINE_SURFACE_WITH_KNOTS((4,4),(3,3),(0.,0.000511815456479786),(0.,1.00105873159848),
 .UNSPECIFIED.)
GEOMETRIC_REPRESENTATION_ITEM()
RATIONAL_B_SPLINE_SURFACE(((1.,0.708394529056752,1.00061746385276),(1.,
0.708058564167294,1.00061817524605),(1.,0.707430835372481,1.00061950443867),
(1.,0.706796685880808,1.00062084722688)))
REPRESENTATION_ITEM('')
SURFACE()
);
#2829=(
BOUNDED_SURFACE()
B_SPLINE_SURFACE(3,2,((#203489,#203490,#203491),(#203492,#203493,#203494),
(#203495,#203496,#203497),(#203498,#203499,#203500)),.UNSPECIFIED.,.F.,
 .F.,.F.)
B_SPLINE_SURFACE_WITH_KNOTS((4,4),(3,3),(0.,0.000397394465448307),(0.,1.),
 .UNSPECIFIED.)
GEOMETRIC_REPRESENTATION_ITEM()
RATIONAL_B_SPLINE_SURFACE(((1.,0.705498956110761,1.),(1.,0.705821764811792,
1.),(1.,0.706461952521129,1.),(1.,0.707106781186548,1.)))
REPRESENTATION_ITEM('')
SURFACE()
);
#2830=(
BOUNDED_SURFACE()
B_SPLINE_SURFACE(3,2,((#203506,#203507,#203508),(#203509,#203510,#203511),
(#203512,#203513,#203514),(#203515,#203516,#203517)),.UNSPECIFIED.,.F.,
 .F.,.F.)
B_SPLINE_SURFACE_WITH_KNOTS((4,4),(3,3),(0.,0.000397394410828738),(0.,1.),
 .UNSPECIFIED.)
GEOMETRIC_REPRESENTATION_ITEM()
RATIONAL_B_SPLINE_SURFACE(((1.,0.708689770883313,1.),(1.,0.708376440034526,
1.),(1.,0.707750498698415,1.),(1.,0.707106781186548,1.)))
REPRESENTATION_ITEM('')
SURFACE()
);
#2831=(
BOUNDED_SURFACE()
B_SPLINE_SURFACE(3,2,((#203523,#203524,#203525),(#203526,#203527,#203528),
(#203529,#203530,#203531),(#203532,#203533,#203534)),.UNSPECIFIED.,.F.,
 .F.,.F.)
B_SPLINE_SURFACE_WITH_KNOTS((4,4),(3,3),(0.,0.000511815090126175),(0.,1.00105592270185),
 .UNSPECIFIED.)
GEOMETRIC_REPRESENTATION_ITEM()
RATIONAL_B_SPLINE_SURFACE(((1.,0.705266242717582,1.00062243213063),(1.,
0.705584085909227,1.00062176089495),(1.,0.706182089450609,1.00062049800392),
(1.,0.70679750858758,1.00061919833384)))
REPRESENTATION_ITEM('')
SURFACE()
);
#2832=(
BOUNDED_SURFACE()
B_SPLINE_SURFACE(3,2,((#203536,#203537,#203538),(#203539,#203540,#203541),
(#203542,#203543,#203544),(#203545,#203546,#203547)),.UNSPECIFIED.,.F.,
 .F.,.F.)
B_SPLINE_SURFACE_WITH_KNOTS((4,4),(3,3),(0.,0.000397394428086637),(0.,1.),
 .UNSPECIFIED.)
GEOMETRIC_REPRESENTATION_ITEM()
RATIONAL_B_SPLINE_SURFACE(((1.,0.707106781186542,1.),(1.,0.706459846759078,
1.),(1.,0.705820510737287,1.),(1.,0.705498956110738,1.)))
REPRESENTATION_ITEM('')
SURFACE()
);
#2833=(
BOUNDED_SURFACE()
B_SPLINE_SURFACE(3,2,((#203553,#203554,#203555),(#203556,#203557,#203558),
(#203559,#203560,#203561),(#203562,#203563,#203564),(#203565,#203566,#203567),
(#203568,#203569,#203570)),.UNSPECIFIED.,.F.,.F.,.F.)
B_SPLINE_SURFACE_WITH_KNOTS((4,2,4),(3,3),(0.,0.000257953807872848,0.000515907615745695),
(0.,1.),.UNSPECIFIED.)
GEOMETRIC_REPRESENTATION_ITEM()
RATIONAL_B_SPLINE_SURFACE(((1.,0.874619707139392,1.),(1.,0.874834349678565,
1.),(1.,0.854686104158367,1.),(1.,0.792476597914559,1.),(1.,0.750887854595556,
1.),(1.,0.705585838031436,1.)))
REPRESENTATION_ITEM('')
SURFACE()
);
#2834=(
BOUNDED_SURFACE()
B_SPLINE_SURFACE(3,2,((#203576,#203577,#203578),(#203579,#203580,#203581),
(#203582,#203583,#203584),(#203585,#203586,#203587)),.UNSPECIFIED.,.F.,
 .F.,.F.)
B_SPLINE_SURFACE_WITH_KNOTS((4,4),(3,3),(0.,0.000511815437699153),(0.,1.00105881331522),
 .UNSPECIFIED.)
GEOMETRIC_REPRESENTATION_ITEM()
RATIONAL_B_SPLINE_SURFACE(((1.,0.706796661946524,1.0006208951968),(1.,0.707430821225403,
1.00061955228422),(1.,0.708058545830954,1.00061822299788),(1.,0.708394505252897,
1.00061751156126)))
REPRESENTATION_ITEM('')
SURFACE()
);
#2835=(
BOUNDED_SURFACE()
B_SPLINE_SURFACE(3,2,((#203589,#203590,#203591),(#203592,#203593,#203594),
(#203595,#203596,#203597),(#203598,#203599,#203600),(#203601,#203602,#203603),
(#203604,#203605,#203606)),.UNSPECIFIED.,.F.,.F.,.F.)
B_SPLINE_SURFACE_WITH_KNOTS((4,2,4),(3,3),(0.,0.000256915317531264,0.000513830635062528),
(0.,1.),.UNSPECIFIED.)
GEOMETRIC_REPRESENTATION_ITEM()
RATIONAL_B_SPLINE_SURFACE(((1.,0.705585838031451,1.),(1.,0.750902433543144,
1.),(1.,0.792329530082004,1.),(1.,0.854288401594724,1.),(1.,0.874998031124746,
1.),(1.,0.87461970713938,1.)))
REPRESENTATION_ITEM('')
SURFACE()
);
#2836=(
BOUNDED_SURFACE()
B_SPLINE_SURFACE(3,2,((#203612,#203613,#203614),(#203615,#203616,#203617),
(#203618,#203619,#203620),(#203621,#203622,#203623),(#203624,#203625,#203626),
(#203627,#203628,#203629)),.UNSPECIFIED.,.F.,.F.,.F.)
B_SPLINE_SURFACE_WITH_KNOTS((4,2,4),(3,3),(-5.77337656848531E-18,0.000256592814262153,
0.000513185628524311),(0.,1.),.UNSPECIFIED.)
GEOMETRIC_REPRESENTATION_ITEM()
RATIONAL_B_SPLINE_SURFACE(((1.,0.708712527163686,1.),(1.,0.753780902613222,
1.),(1.,0.794538995769662,1.),(1.,0.855070770330659,1.),(1.,0.875018427445666,
1.),(1.,0.874619707139391,1.)))
REPRESENTATION_ITEM('')
SURFACE()
);
#2837=(
BOUNDED_SURFACE()
B_SPLINE_SURFACE(3,2,((#203631,#203632,#203633),(#203634,#203635,#203636),
(#203637,#203638,#203639),(#203640,#203641,#203642)),.UNSPECIFIED.,.F.,
 .F.,.F.)
B_SPLINE_SURFACE_WITH_KNOTS((4,4),(3,3),(-6.50521303491303E-18,0.000511815072430408),
(0.,1.00105598365618),.UNSPECIFIED.)
GEOMETRIC_REPRESENTATION_ITEM()
RATIONAL_B_SPLINE_SURFACE(((1.,0.706797490734475,1.00061923411547),(1.,
0.706182062147388,1.00062053388053),(1.,0.705584062769775,1.00062179683567),
(1.,0.705266224771253,1.00062246809913)))
REPRESENTATION_ITEM('')
SURFACE()
);
#2838=(
BOUNDED_SURFACE()
B_SPLINE_SURFACE(3,2,((#203648,#203649,#203650),(#203651,#203652,#203653),
(#203654,#203655,#203656),(#203657,#203658,#203659),(#203660,#203661,#203662),
(#203663,#203664,#203665)),.UNSPECIFIED.,.F.,.F.,.F.)
B_SPLINE_SURFACE_WITH_KNOTS((4,2,4),(3,3),(0.,0.000257652232350882,0.000515304464701765),
(0.,1.),.UNSPECIFIED.)
GEOMETRIC_REPRESENTATION_ITEM()
RATIONAL_B_SPLINE_SURFACE(((1.,0.874619707139388,1.),(1.,0.874861180430391,
1.),(1.,0.855455725921296,1.),(1.,0.794699358954867,1.),(1.,0.753768977788935,
1.),(1.,0.708712527163671,1.)))
REPRESENTATION_ITEM('')
SURFACE()
);
#2839=(
BOUNDED_SURFACE()
B_SPLINE_SURFACE(3,2,((#203671,#203672,#203673),(#203674,#203675,#203676),
(#203677,#203678,#203679),(#203680,#203681,#203682)),.UNSPECIFIED.,.F.,
 .F.,.F.)
B_SPLINE_SURFACE_WITH_KNOTS((4,4),(3,3),(-6.47810798060089E-18,0.000397394373651925),
(0.,1.),.UNSPECIFIED.)
GEOMETRIC_REPRESENTATION_ITEM()
RATIONAL_B_SPLINE_SURFACE(((1.,0.707106781186548,1.),(1.,0.707752587915882,
1.),(1.,0.708377654540684,1.),(1.,0.708689770883318,1.)))
REPRESENTATION_ITEM('')
SURFACE()
);
#2840=(
BOUNDED_SURFACE()
B_SPLINE_SURFACE(3,2,((#203684,#203685,#203686),(#203687,#203688,#203689),
(#203690,#203691,#203692),(#203693,#203694,#203695)),.UNSPECIFIED.,.F.,
 .F.,.F.)
B_SPLINE_SURFACE_WITH_KNOTS((4,4),(3,3),(0.,0.000511815456479792),(0.,1.0010587315997),
 .UNSPECIFIED.)
GEOMETRIC_REPRESENTATION_ITEM()
RATIONAL_B_SPLINE_SURFACE(((1.,0.708394529056393,1.00061746385347),(1.,
0.708058564166965,1.00061817524676),(1.,0.707430835372115,1.00061950443938),
(1.,0.706796685880457,1.00062084722759)))
REPRESENTATION_ITEM('')
SURFACE()
);
#2841=(
BOUNDED_SURFACE()
B_SPLINE_SURFACE(3,2,((#203701,#203702,#203703),(#203704,#203705,#203706),
(#203707,#203708,#203709),(#203710,#203711,#203712)),.UNSPECIFIED.,.F.,
 .F.,.F.)
B_SPLINE_SURFACE_WITH_KNOTS((4,4),(3,3),(-6.50521303491303E-18,0.000397394465448295),
(0.,1.),.UNSPECIFIED.)
GEOMETRIC_REPRESENTATION_ITEM()
RATIONAL_B_SPLINE_SURFACE(((1.,0.705498956110763,1.),(1.,0.705821764811782,
1.),(1.,0.706461952521153,1.),(1.,0.707106781186548,1.)))
REPRESENTATION_ITEM('')
SURFACE()
);
#2842=(
BOUNDED_SURFACE()
B_SPLINE_SURFACE(3,2,((#203718,#203719,#203720),(#203721,#203722,#203723),
(#203724,#203725,#203726),(#203727,#203728,#203729)),.UNSPECIFIED.,.F.,
 .F.,.F.)
B_SPLINE_SURFACE_WITH_KNOTS((4,4),(3,3),(0.,0.000397394410828746),(0.,1.),
 .UNSPECIFIED.)
GEOMETRIC_REPRESENTATION_ITEM()
RATIONAL_B_SPLINE_SURFACE(((1.,0.708689770883334,1.),(1.,0.708376440034459,
1.),(1.,0.707750498698428,1.),(1.,0.707106781186548,1.)))
REPRESENTATION_ITEM('')
SURFACE()
);
#2843=(
BOUNDED_SURFACE()
B_SPLINE_SURFACE(3,2,((#203735,#203736,#203737),(#203738,#203739,#203740),
(#203741,#203742,#203743),(#203744,#203745,#203746)),.UNSPECIFIED.,.F.,
 .F.,.F.)
B_SPLINE_SURFACE_WITH_KNOTS((4,4),(3,3),(0.,0.000511815090126176),(0.,1.00105592270255),
 .UNSPECIFIED.)
GEOMETRIC_REPRESENTATION_ITEM()
RATIONAL_B_SPLINE_SURFACE(((1.,0.705266242717375,1.00062243213105),(1.,
0.705584085909053,1.00062176089536),(1.,0.706182089450385,1.00062049800433),
(1.,0.706797508587384,1.00061919833425)))
REPRESENTATION_ITEM('')
SURFACE()
);
#2844=(
BOUNDED_SURFACE()
B_SPLINE_SURFACE(3,2,((#203748,#203749,#203750),(#203751,#203752,#203753),
(#203754,#203755,#203756),(#203757,#203758,#203759)),.UNSPECIFIED.,.F.,
 .F.,.F.)
B_SPLINE_SURFACE_WITH_KNOTS((4,4),(3,3),(-7.04731412115578E-18,0.000397394428086627),
(0.,1.),.UNSPECIFIED.)
GEOMETRIC_REPRESENTATION_ITEM()
RATIONAL_B_SPLINE_SURFACE(((1.,0.707106781186552,1.),(1.,0.706459846759089,
1.),(1.,0.705820510737279,1.),(1.,0.70549895611075,1.)))
REPRESENTATION_ITEM('')
SURFACE()
);
#2845=(
BOUNDED_SURFACE()
B_SPLINE_SURFACE(3,2,((#203765,#203766,#203767),(#203768,#203769,#203770),
(#203771,#203772,#203773),(#203774,#203775,#203776),(#203777,#203778,#203779),
(#203780,#203781,#203782)),.UNSPECIFIED.,.F.,.F.,.F.)
B_SPLINE_SURFACE_WITH_KNOTS((4,2,4),(3,3),(0.,0.000257953807872837,0.000515907615745675),
(0.,1.),.UNSPECIFIED.)
GEOMETRIC_REPRESENTATION_ITEM()
RATIONAL_B_SPLINE_SURFACE(((1.,0.874619707139391,1.),(1.,0.874834349678828,
1.),(1.,0.854686104158017,1.),(1.,0.792476597914933,1.),(1.,0.750887854595276,
1.),(1.,0.705585838031441,1.)))
REPRESENTATION_ITEM('')
SURFACE()
);
#2846=(
BOUNDED_SURFACE()
B_SPLINE_SURFACE(3,2,((#203788,#203789,#203790),(#203791,#203792,#203793),
(#203794,#203795,#203796),(#203797,#203798,#203799)),.UNSPECIFIED.,.F.,
 .F.,.F.)
B_SPLINE_SURFACE_WITH_KNOTS((4,4),(3,3),(0.,0.000511815437699145),(0.,1.00105881331634),
 .UNSPECIFIED.)
GEOMETRIC_REPRESENTATION_ITEM()
RATIONAL_B_SPLINE_SURFACE(((1.,0.706796661946205,1.00062089519746),(1.,
0.707430821225054,1.00061955228488),(1.,0.708058545830615,1.00061822299854),
(1.,0.708394505252581,1.00061751156192)))
REPRESENTATION_ITEM('')
SURFACE()
);
#2847=(
BOUNDED_SURFACE()
B_SPLINE_SURFACE(3,2,((#203801,#203802,#203803),(#203804,#203805,#203806),
(#203807,#203808,#203809),(#203810,#203811,#203812),(#203813,#203814,#203815),
(#203816,#203817,#203818)),.UNSPECIFIED.,.F.,.F.,.F.)
B_SPLINE_SURFACE_WITH_KNOTS((4,2,4),(3,3),(0.,0.00025691531753126,0.00051383063506252),
(0.,1.),.UNSPECIFIED.)
GEOMETRIC_REPRESENTATION_ITEM()
RATIONAL_B_SPLINE_SURFACE(((1.,0.705585838031456,1.),(1.,0.750902433542903,
1.),(1.,0.792329530082338,1.),(1.,0.854288401594379,1.),(1.,0.874998031125013,
1.),(1.,0.874619707139406,1.)))
REPRESENTATION_ITEM('')
SURFACE()
);
#2848=(
BOUNDED_SURFACE()
B_SPLINE_SURFACE(3,2,((#203824,#203825,#203826),(#203827,#203828,#203829),
(#203830,#203831,#203832),(#203833,#203834,#203835),(#203836,#203837,#203838),
(#203839,#203840,#203841)),.UNSPECIFIED.,.F.,.F.,.F.)
B_SPLINE_SURFACE_WITH_KNOTS((4,2,4),(3,3),(-1.00559751498031E-17,0.000256592814262151,
0.000513185628524312),(0.,1.),.UNSPECIFIED.)
GEOMETRIC_REPRESENTATION_ITEM()
RATIONAL_B_SPLINE_SURFACE(((1.,0.708712527163686,1.),(1.,0.753780902613619,
1.),(1.,0.794538995769145,1.),(1.,0.855070770331154,1.),(1.,0.875018427445275,
1.),(1.,0.874619707139389,1.)))
REPRESENTATION_ITEM('')
SURFACE()
);
#2849=(
BOUNDED_SURFACE()
B_SPLINE_SURFACE(3,2,((#203843,#203844,#203845),(#203846,#203847,#203848),
(#203849,#203850,#203851),(#203852,#203853,#203854)),.UNSPECIFIED.,.F.,
 .F.,.F.)
B_SPLINE_SURFACE_WITH_KNOTS((4,4),(3,3),(0.,0.000511815072430401),(0.,1.00105598365772),
 .UNSPECIFIED.)
GEOMETRIC_REPRESENTATION_ITEM()
RATIONAL_B_SPLINE_SURFACE(((1.,0.706797490734024,1.00061923411637),(1.,
0.706182062146945,1.00062053388144),(1.,0.705584062769309,1.00062179683658),
(1.,0.705266224770789,1.00062246810004)))
REPRESENTATION_ITEM('')
SURFACE()
);
#2850=(
BOUNDED_SURFACE()
B_SPLINE_SURFACE(3,2,((#203860,#203861,#203862),(#203863,#203864,#203865),
(#203866,#203867,#203868),(#203869,#203870,#203871),(#203872,#203873,#203874),
(#203875,#203876,#203877)),.UNSPECIFIED.,.F.,.F.,.F.)
B_SPLINE_SURFACE_WITH_KNOTS((4,2,4),(3,3),(0.,0.000257652232350878,0.000515304464701757),
(0.,1.),.UNSPECIFIED.)
GEOMETRIC_REPRESENTATION_ITEM()
RATIONAL_B_SPLINE_SURFACE(((1.,0.87461970713938,1.),(1.,0.87486118043086,
1.),(1.,0.855455725920641,1.),(1.,0.794699358955482,1.),(1.,0.753768977788477,
1.),(1.,0.708712527163645,1.)))
REPRESENTATION_ITEM('')
SURFACE()
);
#2851=(
BOUNDED_SURFACE()
B_SPLINE_SURFACE(3,2,((#203883,#203884,#203885),(#203886,#203887,#203888),
(#203889,#203890,#203891),(#203892,#203893,#203894)),.UNSPECIFIED.,.F.,
 .F.,.F.)
B_SPLINE_SURFACE_WITH_KNOTS((4,4),(3,3),(0.,0.000397394373651912),(0.,1.),
 .UNSPECIFIED.)
GEOMETRIC_REPRESENTATION_ITEM()
RATIONAL_B_SPLINE_SURFACE(((1.,0.707106781186552,1.),(1.,0.707752587915898,
1.),(1.,0.708377654540669,1.),(1.,0.708689770883344,1.)))
REPRESENTATION_ITEM('')
SURFACE()
);
#2852=(
BOUNDED_SURFACE()
B_SPLINE_SURFACE(3,2,((#203896,#203897,#203898),(#203899,#203900,#203901),
(#203902,#203903,#203904),(#203905,#203906,#203907)),.UNSPECIFIED.,.F.,
 .F.,.F.)
B_SPLINE_SURFACE_WITH_KNOTS((4,4),(3,3),(0.,0.000511815456479782),(0.,1.00105873160036),
 .UNSPECIFIED.)
GEOMETRIC_REPRESENTATION_ITEM()
RATIONAL_B_SPLINE_SURFACE(((1.,0.708394529056206,1.00061746385385),(1.,
0.708058564166767,1.00061817524714),(1.,0.707430835371931,1.00061950443977),
(1.,0.706796685880258,1.00062084722798)))
REPRESENTATION_ITEM('')
SURFACE()
);
#2853=(
BOUNDED_SURFACE()
B_SPLINE_SURFACE(3,2,((#203913,#203914,#203915),(#203916,#203917,#203918),
(#203919,#203920,#203921),(#203922,#203923,#203924)),.UNSPECIFIED.,.F.,
 .F.,.F.)
B_SPLINE_SURFACE_WITH_KNOTS((4,4),(3,3),(0.,0.000397394465448309),(0.,1.),
 .UNSPECIFIED.)
GEOMETRIC_REPRESENTATION_ITEM()
RATIONAL_B_SPLINE_SURFACE(((1.,0.705498956110771,1.),(1.,0.705821764811772,
1.),(1.,0.706461952521137,1.),(1.,0.707106781186542,1.)))
REPRESENTATION_ITEM('')
SURFACE()
);
#2854=(
BOUNDED_SURFACE()
B_SPLINE_SURFACE(3,2,((#203930,#203931,#203932),(#203933,#203934,#203935),
(#203936,#203937,#203938),(#203939,#203940,#203941)),.UNSPECIFIED.,.F.,
 .F.,.F.)
B_SPLINE_SURFACE_WITH_KNOTS((4,4),(3,3),(0.,0.000397394410828738),(0.,1.),
 .UNSPECIFIED.)
GEOMETRIC_REPRESENTATION_ITEM()
RATIONAL_B_SPLINE_SURFACE(((1.,0.708689770883327,1.),(1.,0.708376440034483,
1.),(1.,0.707750498698405,1.),(1.,0.707106781186548,1.)))
REPRESENTATION_ITEM('')
SURFACE()
);
#2855=(
BOUNDED_SURFACE()
B_SPLINE_SURFACE(3,2,((#203947,#203948,#203949),(#203950,#203951,#203952),
(#203953,#203954,#203955),(#203956,#203957,#203958)),.UNSPECIFIED.,.F.,
 .F.,.F.)
B_SPLINE_SURFACE_WITH_KNOTS((4,4),(3,3),(0.,0.000511815090126174),(0.,1.00105592270161),
 .UNSPECIFIED.)
GEOMETRIC_REPRESENTATION_ITEM()
RATIONAL_B_SPLINE_SURFACE(((1.,0.705266242717667,1.00062243213049),(1.,
0.705584085909315,1.0006217608948),(1.,0.706182089450683,1.00062049800377),
(1.,0.706797508587654,1.0006191983337)))
REPRESENTATION_ITEM('')
SURFACE()
);
#2856=(
BOUNDED_SURFACE()
B_SPLINE_SURFACE(3,2,((#203960,#203961,#203962),(#203963,#203964,#203965),
(#203966,#203967,#203968),(#203969,#203970,#203971)),.UNSPECIFIED.,.F.,
 .F.,.F.)
B_SPLINE_SURFACE_WITH_KNOTS((4,4),(3,3),(0.,0.000397394428086627),(0.,1.),
 .UNSPECIFIED.)
GEOMETRIC_REPRESENTATION_ITEM()
RATIONAL_B_SPLINE_SURFACE(((1.,0.707106781186548,1.),(1.,0.706459846759099,
1.),(1.,0.705820510737275,1.),(1.,0.705498956110758,1.)))
REPRESENTATION_ITEM('')
SURFACE()
);
#2857=(
BOUNDED_SURFACE()
B_SPLINE_SURFACE(3,2,((#203977,#203978,#203979),(#203980,#203981,#203982),
(#203983,#203984,#203985),(#203986,#203987,#203988),(#203989,#203990,#203991),
(#203992,#203993,#203994)),.UNSPECIFIED.,.F.,.F.,.F.)
B_SPLINE_SURFACE_WITH_KNOTS((4,2,4),(3,3),(0.,0.00025795380787285,0.000515907615745701),
(0.,1.),.UNSPECIFIED.)
GEOMETRIC_REPRESENTATION_ITEM()
RATIONAL_B_SPLINE_SURFACE(((1.,0.874619707139387,1.),(1.,0.874834349679026,
1.),(1.,0.854686104157727,1.),(1.,0.79247659791521,1.),(1.,0.750887854595059,
1.),(1.,0.705585838031472,1.)))
REPRESENTATION_ITEM('')
SURFACE()
);
#2858=(
BOUNDED_SURFACE()
B_SPLINE_SURFACE(3,2,((#204000,#204001,#204002),(#204003,#204004,#204005),
(#204006,#204007,#204008),(#204009,#204010,#204011)),.UNSPECIFIED.,.F.,
 .F.,.F.)
B_SPLINE_SURFACE_WITH_KNOTS((4,4),(3,3),(-6.91178884959509E-18,0.000511815437699152),
(0.,1.00105881331612),.UNSPECIFIED.)
GEOMETRIC_REPRESENTATION_ITEM()
RATIONAL_B_SPLINE_SURFACE(((1.,0.706796661946268,1.00062089519732),(1.,
0.707430821225128,1.00061955228474),(1.,0.708058545830661,1.0006182229984),
(1.,0.708394505252647,1.00061751156178)))
REPRESENTATION_ITEM('')
SURFACE()
);
#2859=(
BOUNDED_SURFACE()
B_SPLINE_SURFACE(3,2,((#204013,#204014,#204015),(#204016,#204017,#204018),
(#204019,#204020,#204021),(#204022,#204023,#204024),(#204025,#204026,#204027),
(#204028,#204029,#204030)),.UNSPECIFIED.,.F.,.F.,.F.)
B_SPLINE_SURFACE_WITH_KNOTS((4,2,4),(3,3),(0.,0.000256915317531256,0.000513830635062513),
(0.,1.),.UNSPECIFIED.)
GEOMETRIC_REPRESENTATION_ITEM()
RATIONAL_B_SPLINE_SURFACE(((1.,0.705585838031416,1.),(1.,0.750902433543309,
1.),(1.,0.792329530081767,1.),(1.,0.854288401594944,1.),(1.,0.874998031124557,
1.),(1.,0.874619707139388,1.)))
REPRESENTATION_ITEM('')
SURFACE()
);
#2860=(
BOUNDED_SURFACE()
B_SPLINE_SURFACE(3,2,((#204036,#204037,#204038),(#204039,#204040,#204041),
(#204042,#204043,#204044),(#204045,#204046,#204047),(#204048,#204049,#204050),
(#204051,#204052,#204053)),.UNSPECIFIED.,.F.,.F.,.F.)
B_SPLINE_SURFACE_WITH_KNOTS((4,2,4),(3,3),(-9.86623976961809E-18,0.000256592814262151,
0.000513185628524311),(0.,1.),.UNSPECIFIED.)
GEOMETRIC_REPRESENTATION_ITEM()
RATIONAL_B_SPLINE_SURFACE(((1.,0.708712527163674,1.),(1.,0.753780902613021,
1.),(1.,0.794538995769931,1.),(1.,0.855070770330375,1.),(1.,0.875018427445861,
1.),(1.,0.874619707139398,1.)))
REPRESENTATION_ITEM('')
SURFACE()
);
#2861=(
BOUNDED_SURFACE()
B_SPLINE_SURFACE(3,2,((#204055,#204056,#204057),(#204058,#204059,#204060),
(#204061,#204062,#204063),(#204064,#204065,#204066)),.UNSPECIFIED.,.F.,
 .F.,.F.)
B_SPLINE_SURFACE_WITH_KNOTS((4,4),(3,3),(0.,0.000511815072430404),(0.,1.00105598365858),
 .UNSPECIFIED.)
GEOMETRIC_REPRESENTATION_ITEM()
RATIONAL_B_SPLINE_SURFACE(((1.,0.706797490733775,1.00061923411688),(1.,
0.706182062146654,1.00062053388194),(1.,0.705584062769082,1.00062179683708),
(1.,0.70526622477053,1.00062246810054)))
REPRESENTATION_ITEM('')
SURFACE()
);
#2862=(
BOUNDED_SURFACE()
B_SPLINE_SURFACE(3,2,((#204072,#204073,#204074),(#204075,#204076,#204077),
(#204078,#204079,#204080),(#204081,#204082,#204083),(#204084,#204085,#204086),
(#204087,#204088,#204089)),.UNSPECIFIED.,.F.,.F.,.F.)
B_SPLINE_SURFACE_WITH_KNOTS((4,2,4),(3,3),(-1.68051336735253E-18,0.000257652232350876,
0.000515304464701754),(0.,1.),.UNSPECIFIED.)
GEOMETRIC_REPRESENTATION_ITEM()
RATIONAL_B_SPLINE_SURFACE(((1.,0.874619707139403,1.),(1.,0.874861180431004,
1.),(1.,0.855455725920461,1.),(1.,0.794699358955677,1.),(1.,0.753768977788352,
1.),(1.,0.708712527163669,1.)))
REPRESENTATION_ITEM('')
SURFACE()
);
#2863=(
BOUNDED_SURFACE()
B_SPLINE_SURFACE(3,2,((#204095,#204096,#204097),(#204098,#204099,#204100),
(#204101,#204102,#204103),(#204104,#204105,#204106)),.UNSPECIFIED.,.F.,
 .F.,.F.)
B_SPLINE_SURFACE_WITH_KNOTS((4,4),(3,3),(2.71050543121376E-20,0.000397394373651921),
(0.,1.),.UNSPECIFIED.)
GEOMETRIC_REPRESENTATION_ITEM()
RATIONAL_B_SPLINE_SURFACE(((1.,0.707106781186548,1.),(1.,0.707752587915894,
1.),(1.,0.708377654540691,1.),(1.,0.708689770883335,1.)))
REPRESENTATION_ITEM('')
SURFACE()
);
#2864=(
BOUNDED_SURFACE()
B_SPLINE_SURFACE(3,2,((#204108,#204109,#204110),(#204111,#204112,#204113),
(#204114,#204115,#204116),(#204117,#204118,#204119)),.UNSPECIFIED.,.F.,
 .F.,.F.)
B_SPLINE_SURFACE_WITH_KNOTS((4,4),(3,3),(0.,0.000511815456479785),(0.,1.00105873159947),
 .UNSPECIFIED.)
GEOMETRIC_REPRESENTATION_ITEM()
RATIONAL_B_SPLINE_SURFACE(((1.,0.708394529056476,1.00061746385333),(1.,
0.708058564167017,1.00061817524662),(1.,0.707430835372211,1.00061950443924),
(1.,0.70679668588052,1.00062084722745)))
REPRESENTATION_ITEM('')
SURFACE()
);
#2865=(
BOUNDED_SURFACE()
B_SPLINE_SURFACE(3,2,((#204125,#204126,#204127),(#204128,#204129,#204130),
(#204131,#204132,#204133),(#204134,#204135,#204136)),.UNSPECIFIED.,.F.,
 .F.,.F.)
B_SPLINE_SURFACE_WITH_KNOTS((4,4),(3,3),(0.,0.00039739446544831),(0.,1.),
 .UNSPECIFIED.)
GEOMETRIC_REPRESENTATION_ITEM()
RATIONAL_B_SPLINE_SURFACE(((1.,0.705498956110746,1.),(1.,0.705821764811779,
1.),(1.,0.706461952521139,1.),(1.,0.707106781186548,1.)))
REPRESENTATION_ITEM('')
SURFACE()
);
#2866=(
BOUNDED_SURFACE()
B_SPLINE_SURFACE(3,2,((#204142,#204143,#204144),(#204145,#204146,#204147),
(#204148,#204149,#204150),(#204151,#204152,#204153)),.UNSPECIFIED.,.F.,
 .F.,.F.)
B_SPLINE_SURFACE_WITH_KNOTS((4,4),(3,3),(0.,0.000397394410828733),(0.,1.),
 .UNSPECIFIED.)
GEOMETRIC_REPRESENTATION_ITEM()
RATIONAL_B_SPLINE_SURFACE(((1.,0.708689770883331,1.),(1.,0.708376440034489,
1.),(1.,0.707750498698411,1.),(1.,0.707106781186548,1.)))
REPRESENTATION_ITEM('')
SURFACE()
);
#2867=(
BOUNDED_SURFACE()
B_SPLINE_SURFACE(3,2,((#204159,#204160,#204161),(#204162,#204163,#204164),
(#204165,#204166,#204167),(#204168,#204169,#204170)),.UNSPECIFIED.,.F.,
 .F.,.F.)
B_SPLINE_SURFACE_WITH_KNOTS((4,4),(3,3),(0.,0.000511815090126173),(0.,1.00105592270321),
 .UNSPECIFIED.)
GEOMETRIC_REPRESENTATION_ITEM()
RATIONAL_B_SPLINE_SURFACE(((1.,0.705266242717188,1.00062243213143),(1.,
0.705584085908842,1.00062176089575),(1.,0.706182089450201,1.00062049800472),
(1.,0.706797508587187,1.00061919833464)))
REPRESENTATION_ITEM('')
SURFACE()
);
#2868=(
BOUNDED_SURFACE()
B_SPLINE_SURFACE(3,2,((#204172,#204173,#204174),(#204175,#204176,#204177),
(#204178,#204179,#204180),(#204181,#204182,#204183)),.UNSPECIFIED.,.F.,
 .F.,.F.)
B_SPLINE_SURFACE_WITH_KNOTS((4,4),(3,3),(-6.85757874097082E-18,0.00039739442808662),
(0.,1.),.UNSPECIFIED.)
GEOMETRIC_REPRESENTATION_ITEM()
RATIONAL_B_SPLINE_SURFACE(((1.,0.707106781186548,1.),(1.,0.706459846759094,
1.),(1.,0.705820510737267,1.),(1.,0.705498956110752,1.)))
REPRESENTATION_ITEM('')
SURFACE()
);
#2869=(
BOUNDED_SURFACE()
B_SPLINE_SURFACE(3,2,((#204189,#204190,#204191),(#204192,#204193,#204194),
(#204195,#204196,#204197),(#204198,#204199,#204200),(#204201,#204202,#204203),
(#204204,#204205,#204206)),.UNSPECIFIED.,.F.,.F.,.F.)
B_SPLINE_SURFACE_WITH_KNOTS((4,2,4),(3,3),(0.,0.000257953807872842,0.000515907615745685),
(0.,1.),.UNSPECIFIED.)
GEOMETRIC_REPRESENTATION_ITEM()
RATIONAL_B_SPLINE_SURFACE(((1.,0.874619707139392,1.),(1.,0.874834349678954,
1.),(1.,0.854686104157838,1.),(1.,0.792476597915099,1.),(1.,0.750887854595166,
1.),(1.,0.705585838031451,1.)))
REPRESENTATION_ITEM('')
SURFACE()
);
#2870=(
BOUNDED_SURFACE()
B_SPLINE_SURFACE(3,2,((#204209,#204210,#204211),(#204212,#204213,#204214),
(#204215,#204216,#204217),(#204218,#204219,#204220)),.UNSPECIFIED.,.F.,
 .F.,.F.)
B_SPLINE_SURFACE_WITH_KNOTS((4,4),(3,3),(0.,0.000511815437699147),(0.,1.0010588133146),
 .UNSPECIFIED.)
GEOMETRIC_REPRESENTATION_ITEM()
RATIONAL_B_SPLINE_SURFACE(((1.,0.706796661946711,1.00062089519643),(1.,
0.707430821225589,1.00061955228386),(1.,0.708058545831085,1.00061822299752),
(1.,0.70839450525309,1.0006175115609)))
REPRESENTATION_ITEM('')
SURFACE()
);
#2871=(
BOUNDED_SURFACE()
B_SPLINE_SURFACE(3,2,((#204222,#204223,#204224),(#204225,#204226,#204227),
(#204228,#204229,#204230),(#204231,#204232,#204233),(#204234,#204235,#204236),
(#204237,#204238,#204239)),.UNSPECIFIED.,.F.,.F.,.F.)
B_SPLINE_SURFACE_WITH_KNOTS((4,2,4),(3,3),(0.,0.000256915317531259,0.000513830635062518),
(0.,1.),.UNSPECIFIED.)
GEOMETRIC_REPRESENTATION_ITEM()
RATIONAL_B_SPLINE_SURFACE(((1.,0.705585838031441,1.),(1.,0.750902433542931,
1.),(1.,0.79232953008227,1.),(1.,0.854288401594435,1.),(1.,0.874998031124952,
1.),(1.,0.874619707139392,1.)))
REPRESENTATION_ITEM('')
SURFACE()
);
#2872=(
BOUNDED_SURFACE()
B_SPLINE_SURFACE(3,2,((#204245,#204246,#204247),(#204248,#204249,#204250),
(#204251,#204252,#204253),(#204254,#204255,#204256),(#204257,#204258,#204259),
(#204260,#204261,#204262)),.UNSPECIFIED.,.F.,.F.,.F.)
B_SPLINE_SURFACE_WITH_KNOTS((4,2,4),(3,3),(-1.56396163381034E-17,0.000256592814262148,
0.000513185628524312),(0.,1.),.UNSPECIFIED.)
GEOMETRIC_REPRESENTATION_ITEM()
RATIONAL_B_SPLINE_SURFACE(((1.,0.708712527163647,1.),(1.,0.753780902613552,
1.),(1.,0.794538995769242,1.),(1.,0.85507077033107,1.),(1.,0.875018427445344,
1.),(1.,0.87461970713939,1.)))
REPRESENTATION_ITEM('')
SURFACE()
);
#2873=(
BOUNDED_SURFACE()
B_SPLINE_SURFACE(3,2,((#204263,#204264,#204265),(#204266,#204267,#204268),
(#204269,#204270,#204271),(#204272,#204273,#204274)),.UNSPECIFIED.,.F.,
 .F.,.F.)
B_SPLINE_SURFACE_WITH_KNOTS((4,4),(3,3),(2.71050543121376E-20,0.000511815072430402),
(0.,1.00105598365742),.UNSPECIFIED.)
GEOMETRIC_REPRESENTATION_ITEM()
RATIONAL_B_SPLINE_SURFACE(((1.,0.706797490734113,1.0006192341162),(1.,0.706182062147032,
1.00062053388126),(1.,0.705584062769394,1.0006217968364),(1.,0.705266224770875,
1.00062246809986)))
REPRESENTATION_ITEM('')
SURFACE()
);
#2874=(
BOUNDED_SURFACE()
B_SPLINE_SURFACE(3,2,((#204278,#204279,#204280),(#204281,#204282,#204283),
(#204284,#204285,#204286),(#204287,#204288,#204289),(#204290,#204291,#204292),
(#204293,#204294,#204295)),.UNSPECIFIED.,.F.,.F.,.F.)
B_SPLINE_SURFACE_WITH_KNOTS((4,2,4),(3,3),(0.,0.000257652232350872,0.000515304464701744),
(0.,1.),.UNSPECIFIED.)
GEOMETRIC_REPRESENTATION_ITEM()
RATIONAL_B_SPLINE_SURFACE(((1.,0.874619707139396,1.),(1.,0.874861180430454,
1.),(1.,0.855455725921202,1.),(1.,0.794699358954921,1.),(1.,0.753768977788908,
1.),(1.,0.708712527163673,1.)))
REPRESENTATION_ITEM('')
SURFACE()
);
#2875=(
BOUNDED_SURFACE()
B_SPLINE_SURFACE(3,2,((#204301,#204302,#204303),(#204304,#204305,#204306),
(#204307,#204308,#204309),(#204310,#204311,#204312)),.UNSPECIFIED.,.F.,
 .F.,.F.)
B_SPLINE_SURFACE_WITH_KNOTS((4,4),(3,3),(0.,0.000397394373651912),(0.,1.),
 .UNSPECIFIED.)
GEOMETRIC_REPRESENTATION_ITEM()
RATIONAL_B_SPLINE_SURFACE(((1.,0.707106781186548,1.),(1.,0.707752587915902,
1.),(1.,0.708377654540677,1.),(1.,0.708689770883331,1.)))
REPRESENTATION_ITEM('')
SURFACE()
);
#2876=(
BOUNDED_SURFACE()
B_SPLINE_SURFACE(3,2,((#204314,#204315,#204316),(#204317,#204318,#204319),
(#204320,#204321,#204322),(#204323,#204324,#204325)),.UNSPECIFIED.,.F.,
 .F.,.F.)
B_SPLINE_SURFACE_WITH_KNOTS((4,4),(3,3),(-6.42389787197661E-18,0.000511815456479786),
(0.,1.00105873159963),.UNSPECIFIED.)
GEOMETRIC_REPRESENTATION_ITEM()
RATIONAL_B_SPLINE_SURFACE(((1.,0.708394529056421,1.00061746385343),(1.,
0.708058564166972,1.00061817524672),(1.,0.707430835372151,1.00061950443934),
(1.,0.706796685880471,1.00062084722755)))
REPRESENTATION_ITEM('')
SURFACE()
);
#2877=(
BOUNDED_SURFACE()
B_SPLINE_SURFACE(3,2,((#204331,#204332,#204333),(#204334,#204335,#204336),
(#204337,#204338,#204339),(#204340,#204341,#204342)),.UNSPECIFIED.,.F.,
 .F.,.F.)
B_SPLINE_SURFACE_WITH_KNOTS((4,4),(3,3),(0.,0.000397394465448313),(0.,1.),
 .UNSPECIFIED.)
GEOMETRIC_REPRESENTATION_ITEM()
RATIONAL_B_SPLINE_SURFACE(((1.,0.705498956110752,1.),(1.,0.705821764811779,
1.),(1.,0.706461952521144,1.),(1.,0.707106781186548,1.)))
REPRESENTATION_ITEM('')
SURFACE()
);
#2878=(
BOUNDED_SURFACE()
B_SPLINE_SURFACE(3,2,((#204348,#204349,#204350),(#204351,#204352,#204353),
(#204354,#204355,#204356),(#204357,#204358,#204359)),.UNSPECIFIED.,.F.,
 .F.,.F.)
B_SPLINE_SURFACE_WITH_KNOTS((4,4),(3,3),(0.,0.000397394410828731),(0.,1.),
 .UNSPECIFIED.)
GEOMETRIC_REPRESENTATION_ITEM()
RATIONAL_B_SPLINE_SURFACE(((1.,0.708689770883323,1.),(1.,0.708376440034485,
1.),(1.,0.707750498698409,1.),(1.,0.707106781186548,1.)))
REPRESENTATION_ITEM('')
SURFACE()
);
#2879=(
BOUNDED_SURFACE()
B_SPLINE_SURFACE(3,2,((#204365,#204366,#204367),(#204368,#204369,#204370),
(#204371,#204372,#204373),(#204374,#204375,#204376)),.UNSPECIFIED.,.F.,
 .F.,.F.)
B_SPLINE_SURFACE_WITH_KNOTS((4,4),(3,3),(0.,0.000511815090126173),(0.,1.00105592270208),
 .UNSPECIFIED.)
GEOMETRIC_REPRESENTATION_ITEM()
RATIONAL_B_SPLINE_SURFACE(((1.,0.705266242717525,1.00062243213077),(1.,
0.705584085909185,1.00062176089509),(1.,0.70618208945054,1.00062049800406),
(1.,0.706797508587514,1.00061919833398)))
REPRESENTATION_ITEM('')
SURFACE()
);
#2880=(
BOUNDED_SURFACE()
B_SPLINE_SURFACE(3,2,((#204378,#204379,#204380),(#204381,#204382,#204383),
(#204384,#204385,#204386),(#204387,#204388,#204389)),.UNSPECIFIED.,.F.,
 .F.,.F.)
B_SPLINE_SURFACE_WITH_KNOTS((4,4),(3,3),(-6.88468379528295E-18,0.000397394428086624),
(0.,1.),.UNSPECIFIED.)
GEOMETRIC_REPRESENTATION_ITEM()
RATIONAL_B_SPLINE_SURFACE(((1.,0.707106781186548,1.),(1.,0.706459846759089,
1.),(1.,0.705820510737284,1.),(1.,0.705498956110758,1.)))
REPRESENTATION_ITEM('')
SURFACE()
);
#2881=(
BOUNDED_SURFACE()
B_SPLINE_SURFACE(3,2,((#204395,#204396,#204397),(#204398,#204399,#204400),
(#204401,#204402,#204403),(#204404,#204405,#204406),(#204407,#204408,#204409),
(#204410,#204411,#204412)),.UNSPECIFIED.,.F.,.F.,.F.)
B_SPLINE_SURFACE_WITH_KNOTS((4,2,4),(3,3),(-8.53809210832335E-19,0.000257953807872841,
0.000515907615745682),(0.,1.),.UNSPECIFIED.)
GEOMETRIC_REPRESENTATION_ITEM()
RATIONAL_B_SPLINE_SURFACE(((1.,0.874619707139387,1.),(1.,0.874834349679282,
1.),(1.,0.854686104157425,1.),(1.,0.792476597915532,1.),(1.,0.750887854594857,
1.),(1.,0.705585838031449,1.)))
REPRESENTATION_ITEM('')
SURFACE()
);
#2882=(
BOUNDED_SURFACE()
B_SPLINE_SURFACE(3,2,((#204418,#204419,#204420),(#204421,#204422,#204423),
(#204424,#204425,#204426),(#204427,#204428,#204429)),.UNSPECIFIED.,.F.,
 .F.,.F.)
B_SPLINE_SURFACE_WITH_KNOTS((4,4),(3,3),(0.,0.000511815437699153),(0.,1.00105881331446),
 .UNSPECIFIED.)
GEOMETRIC_REPRESENTATION_ITEM()
RATIONAL_B_SPLINE_SURFACE(((1.,0.706796661946756,1.00062089519635),(1.,
0.707430821225617,1.00061955228377),(1.,0.708058545831129,1.00061822299743),
(1.,0.708394505253124,1.00061751156081)))
REPRESENTATION_ITEM('')
SURFACE()
);
#2883=(
BOUNDED_SURFACE()
B_SPLINE_SURFACE(3,2,((#204431,#204432,#204433),(#204434,#204435,#204436),
(#204437,#204438,#204439),(#204440,#204441,#204442),(#204443,#204444,#204445),
(#204446,#204447,#204448)),.UNSPECIFIED.,.F.,.F.,.F.)
B_SPLINE_SURFACE_WITH_KNOTS((4,2,4),(3,3),(0.,0.000256915317531263,0.000513830635062527),
(0.,1.),.UNSPECIFIED.)
GEOMETRIC_REPRESENTATION_ITEM()
RATIONAL_B_SPLINE_SURFACE(((1.,0.705585838031433,1.),(1.,0.750902433542847,
1.),(1.,0.792329530082374,1.),(1.,0.85428840159432,1.),(1.,0.87499803112506,
1.),(1.,0.874619707139386,1.)))
REPRESENTATION_ITEM('')
SURFACE()
);
#2884=(
BOUNDED_SURFACE()
B_SPLINE_SURFACE(3,2,((#204454,#204455,#204456),(#204457,#204458,#204459),
(#204460,#204461,#204462),(#204463,#204464,#204465),(#204466,#204467,#204468),
(#204469,#204470,#204471)),.UNSPECIFIED.,.F.,.F.,.F.)
B_SPLINE_SURFACE_WITH_KNOTS((4,2,4),(3,3),(-9.62229428080885E-18,0.000256592814262152,
0.000513185628524313),(0.,1.),.UNSPECIFIED.)
GEOMETRIC_REPRESENTATION_ITEM()
RATIONAL_B_SPLINE_SURFACE(((1.,0.708712527163657,1.),(1.,0.753780902613763,
1.),(1.,0.794538995768959,1.),(1.,0.85507077033135,1.),(1.,0.875018427445137,
1.),(1.,0.87461970713939,1.)))
REPRESENTATION_ITEM('')
SURFACE()
);
#2885=(
BOUNDED_SURFACE()
B_SPLINE_SURFACE(3,2,((#204473,#204474,#204475),(#204476,#204477,#204478),
(#204479,#204480,#204481),(#204482,#204483,#204484)),.UNSPECIFIED.,.F.,
 .F.,.F.)
B_SPLINE_SURFACE_WITH_KNOTS((4,4),(3,3),(-6.91178884959509E-18,0.000511815072430389),
(0.,1.00105598365609),.UNSPECIFIED.)
GEOMETRIC_REPRESENTATION_ITEM()
RATIONAL_B_SPLINE_SURFACE(((1.,0.706797490734499,1.00061923411542),(1.,
0.706182062147426,1.00062053388047),(1.,0.705584062769778,1.00062179683561),
(1.,0.70526622477126,1.00062246809908)))
REPRESENTATION_ITEM('')
SURFACE()
);
#2886=(
BOUNDED_SURFACE()
B_SPLINE_SURFACE(3,2,((#204490,#204491,#204492),(#204493,#204494,#204495),
(#204496,#204497,#204498),(#204499,#204500,#204501),(#204502,#204503,#204504),
(#204505,#204506,#204507)),.UNSPECIFIED.,.F.,.F.,.F.)
B_SPLINE_SURFACE_WITH_KNOTS((4,2,4),(3,3),(-2.57498015965307E-18,0.000257652232350874,
0.000515304464701751),(0.,1.),.UNSPECIFIED.)
GEOMETRIC_REPRESENTATION_ITEM()
RATIONAL_B_SPLINE_SURFACE(((1.,0.874619707139391,1.),(1.,0.874861180430997,
1.),(1.,0.855455725920457,1.),(1.,0.794699358955682,1.),(1.,0.753768977788335,
1.),(1.,0.708712527163661,1.)))
REPRESENTATION_ITEM('')
SURFACE()
);
#2887=(
BOUNDED_SURFACE()
B_SPLINE_SURFACE(3,2,((#204513,#204514,#204515),(#204516,#204517,#204518),
(#204519,#204520,#204521),(#204522,#204523,#204524)),.UNSPECIFIED.,.F.,
 .F.,.F.)
B_SPLINE_SURFACE_WITH_KNOTS((4,4),(3,3),(-6.88468379528295E-18,0.000397394373651904),
(0.,1.),.UNSPECIFIED.)
GEOMETRIC_REPRESENTATION_ITEM()
RATIONAL_B_SPLINE_SURFACE(((1.,0.707106781186548,1.),(1.,0.707752587915922,
1.),(1.,0.708377654540658,1.),(1.,0.708689770883355,1.)))
REPRESENTATION_ITEM('')
SURFACE()
);
#2888=(
BOUNDED_SURFACE()
B_SPLINE_SURFACE(3,2,((#204526,#204527,#204528),(#204529,#204530,#204531),
(#204532,#204533,#204534),(#204535,#204536,#204537)),.UNSPECIFIED.,.F.,
 .F.,.F.)
B_SPLINE_SURFACE_WITH_KNOTS((4,4),(3,3),(0.,0.000511815456479787),(0.,1.00105873160033),
 .UNSPECIFIED.)
GEOMETRIC_REPRESENTATION_ITEM()
RATIONAL_B_SPLINE_SURFACE(((1.,0.708394529056224,1.00061746385383),(1.,
0.708058564166761,1.00061817524712),(1.,0.707430835371962,1.00061950443975),
(1.,0.70679668588027,1.00062084722796)))
REPRESENTATION_ITEM('')
SURFACE()
);
#2889=(
BOUNDED_SURFACE()
B_SPLINE_SURFACE(3,2,((#204543,#204544,#204545),(#204546,#204547,#204548),
(#204549,#204550,#204551),(#204552,#204553,#204554)),.UNSPECIFIED.,.F.,
 .F.,.F.)
B_SPLINE_SURFACE_WITH_KNOTS((4,4),(3,3),(0.,0.00039739446544831),(0.,1.),
 .UNSPECIFIED.)
GEOMETRIC_REPRESENTATION_ITEM()
RATIONAL_B_SPLINE_SURFACE(((1.,0.705498956110744,1.),(1.,0.705821764811777,
1.),(1.,0.706461952521137,1.),(1.,0.70710678118655,1.)))
REPRESENTATION_ITEM('')
SURFACE()
);
#2890=(
BOUNDED_SURFACE()
B_SPLINE_SURFACE(3,2,((#204560,#204561,#204562),(#204563,#204564,#204565),
(#204566,#204567,#204568),(#204569,#204570,#204571)),.UNSPECIFIED.,.F.,
 .F.,.F.)
B_SPLINE_SURFACE_WITH_KNOTS((4,4),(3,3),(0.,0.000397394410828739),(0.,1.),
 .UNSPECIFIED.)
GEOMETRIC_REPRESENTATION_ITEM()
RATIONAL_B_SPLINE_SURFACE(((1.,0.708689770883332,1.),(1.,0.708376440034481,
1.),(1.,0.707750498698418,1.),(1.,0.707106781186543,1.)))
REPRESENTATION_ITEM('')
SURFACE()
);
#2891=(
BOUNDED_SURFACE()
B_SPLINE_SURFACE(3,2,((#204577,#204578,#204579),(#204580,#204581,#204582),
(#204583,#204584,#204585),(#204586,#204587,#204588)),.UNSPECIFIED.,.F.,
 .F.,.F.)
B_SPLINE_SURFACE_WITH_KNOTS((4,4),(3,3),(0.,0.000511815090126177),(0.,1.00105592270103),
 .UNSPECIFIED.)
GEOMETRIC_REPRESENTATION_ITEM()
RATIONAL_B_SPLINE_SURFACE(((1.,0.705266242717828,1.00062243213015),(1.,
0.705584085909493,1.00062176089446),(1.,0.706182089450846,1.00062049800343),
(1.,0.706797508587826,1.00061919833336)))
REPRESENTATION_ITEM('')
SURFACE()
);
#2892=(
BOUNDED_SURFACE()
B_SPLINE_SURFACE(3,2,((#204590,#204591,#204592),(#204593,#204594,#204595),
(#204596,#204597,#204598),(#204599,#204600,#204601)),.UNSPECIFIED.,.F.,
 .F.,.F.)
B_SPLINE_SURFACE_WITH_KNOTS((4,4),(3,3),(0.,0.000397394428086622),(0.,1.),
 .UNSPECIFIED.)
GEOMETRIC_REPRESENTATION_ITEM()
RATIONAL_B_SPLINE_SURFACE(((1.,0.707106781186548,1.),(1.,0.706459846759115,
1.),(1.,0.705820510737262,1.),(1.,0.705498956110746,1.)))
REPRESENTATION_ITEM('')
SURFACE()
);
#2893=(
BOUNDED_SURFACE()
B_SPLINE_SURFACE(3,2,((#204607,#204608,#204609),(#204610,#204611,#204612),
(#204613,#204614,#204615),(#204616,#204617,#204618),(#204619,#204620,#204621),
(#204622,#204623,#204624)),.UNSPECIFIED.,.F.,.F.,.F.)
B_SPLINE_SURFACE_WITH_KNOTS((4,2,4),(3,3),(0.,0.000257953807872836,0.000515907615745673),
(0.,1.),.UNSPECIFIED.)
GEOMETRIC_REPRESENTATION_ITEM()
RATIONAL_B_SPLINE_SURFACE(((1.,0.874619707139392,1.),(1.,0.874834349679114,
1.),(1.,0.854686104157613,1.),(1.,0.792476597915356,1.),(1.,0.750887854594963,
1.),(1.,0.70558583803145,1.)))
REPRESENTATION_ITEM('')
SURFACE()
);
#2894=(
BOUNDED_SURFACE()
B_SPLINE_SURFACE(3,2,((#204630,#204631,#204632),(#204633,#204634,#204635),
(#204636,#204637,#204638),(#204639,#204640,#204641)),.UNSPECIFIED.,.F.,
 .F.,.F.)
B_SPLINE_SURFACE_WITH_KNOTS((4,4),(3,3),(0.,0.000511815437699158),(0.,1.00105881331778),
 .UNSPECIFIED.)
GEOMETRIC_REPRESENTATION_ITEM()
RATIONAL_B_SPLINE_SURFACE(((1.,0.70679666194578,1.0006208951983),(1.,0.707430821224659,
1.00061955228572),(1.,0.708058545830176,1.00061822299938),(1.,0.708394505252165,
1.00061751156276)))
REPRESENTATION_ITEM('')
SURFACE()
);
#2895=(
BOUNDED_SURFACE()
B_SPLINE_SURFACE(3,2,((#204643,#204644,#204645),(#204646,#204647,#204648),
(#204649,#204650,#204651),(#204652,#204653,#204654),(#204655,#204656,#204657),
(#204658,#204659,#204660)),.UNSPECIFIED.,.F.,.F.,.F.)
B_SPLINE_SURFACE_WITH_KNOTS((4,2,4),(3,3),(0.,0.000256915317531259,0.000513830635062518),
(0.,1.),.UNSPECIFIED.)
GEOMETRIC_REPRESENTATION_ITEM()
RATIONAL_B_SPLINE_SURFACE(((1.,0.70558583803145,1.),(1.,0.750902433543056,
1.),(1.,0.792329530082105,1.),(1.,0.854288401594614,1.),(1.,0.874998031124823,
1.),(1.,0.874619707139391,1.)))
REPRESENTATION_ITEM('')
SURFACE()
);
#2896=(
BOUNDED_SURFACE()
B_SPLINE_SURFACE(3,2,((#204666,#204667,#204668),(#204669,#204670,#204671),
(#204672,#204673,#204674),(#204675,#204676,#204677),(#204678,#204679,#204680),
(#204681,#204682,#204683)),.UNSPECIFIED.,.F.,.F.,.F.)
B_SPLINE_SURFACE_WITH_KNOTS((4,2,4),(3,3),(0.,0.000256592814262161,0.000513185628524321),
(0.,1.),.UNSPECIFIED.)
GEOMETRIC_REPRESENTATION_ITEM()
RATIONAL_B_SPLINE_SURFACE(((1.,0.708712527163666,1.),(1.,0.753780902613519,
1.),(1.,0.794538995769293,1.),(1.,0.855070770331016,1.),(1.,0.875018427445383,
1.),(1.,0.874619707139399,1.)))
REPRESENTATION_ITEM('')
SURFACE()
);
#2897=(
BOUNDED_SURFACE()
B_SPLINE_SURFACE(3,2,((#204685,#204686,#204687),(#204688,#204689,#204690),
(#204691,#204692,#204693),(#204694,#204695,#204696)),.UNSPECIFIED.,.F.,
 .F.,.F.)
B_SPLINE_SURFACE_WITH_KNOTS((4,4),(3,3),(0.,0.000511815072430401),(0.,1.0010559836559),
 .UNSPECIFIED.)
GEOMETRIC_REPRESENTATION_ITEM()
RATIONAL_B_SPLINE_SURFACE(((1.,0.706797490734558,1.0006192341153),(1.,0.706182062147484,
1.00062053388036),(1.,0.705584062769846,1.0006217968355),(1.,0.705266224771326,
1.00062246809896)))
REPRESENTATION_ITEM('')
SURFACE()
);
#2898=(
BOUNDED_SURFACE()
B_SPLINE_SURFACE(3,2,((#204702,#204703,#204704),(#204705,#204706,#204707),
(#204708,#204709,#204710),(#204711,#204712,#204713),(#204714,#204715,#204716),
(#204717,#204718,#204719)),.UNSPECIFIED.,.F.,.F.,.F.)
B_SPLINE_SURFACE_WITH_KNOTS((4,2,4),(3,3),(-3.40168431617327E-18,0.000257652232350873,
0.000515304464701749),(0.,1.),.UNSPECIFIED.)
GEOMETRIC_REPRESENTATION_ITEM()
RATIONAL_B_SPLINE_SURFACE(((1.,0.874619707139389,1.),(1.,0.874861180430379,
1.),(1.,0.8554557259213,1.),(1.,0.794699358954817,1.),(1.,0.753768977788956,
1.),(1.,0.70871252716369,1.)))
REPRESENTATION_ITEM('')
SURFACE()
);
#2899=(
BOUNDED_SURFACE()
B_SPLINE_SURFACE(3,2,((#204725,#204726,#204727),(#204728,#204729,#204730),
(#204731,#204732,#204733),(#204734,#204735,#204736)),.UNSPECIFIED.,.F.,
 .F.,.F.)
B_SPLINE_SURFACE_WITH_KNOTS((4,4),(3,3),(0.,0.000397394373651924),(0.,1.),
 .UNSPECIFIED.)
GEOMETRIC_REPRESENTATION_ITEM()
RATIONAL_B_SPLINE_SURFACE(((1.,0.707106781186548,1.),(1.,0.7077525879159,
1.),(1.,0.708377654540681,1.),(1.,0.708689770883329,1.)))
REPRESENTATION_ITEM('')
SURFACE()
);
#2900=(
BOUNDED_SURFACE()
B_SPLINE_SURFACE(3,2,((#204738,#204739,#204740),(#204741,#204742,#204743),
(#204744,#204745,#204746),(#204747,#204748,#204749)),.UNSPECIFIED.,.F.,
 .F.,.F.)
B_SPLINE_SURFACE_WITH_KNOTS((4,4),(3,3),(0.,0.000511815456479784),(0.,1.00105873159911),
 .UNSPECIFIED.)
GEOMETRIC_REPRESENTATION_ITEM()
RATIONAL_B_SPLINE_SURFACE(((1.,0.708394529056574,1.00061746385312),(1.,
0.708058564167126,1.00061817524641),(1.,0.707430835372308,1.00061950443903),
(1.,0.706796685880624,1.00062084722724)))
REPRESENTATION_ITEM('')
SURFACE()
);
#2901=(
BOUNDED_SURFACE()
B_SPLINE_SURFACE(3,2,((#204755,#204756,#204757),(#204758,#204759,#204760),
(#204761,#204762,#204763),(#204764,#204765,#204766)),.UNSPECIFIED.,.F.,
 .F.,.F.)
B_SPLINE_SURFACE_WITH_KNOTS((4,4),(3,3),(0.,0.000397394465448322),(0.,1.),
 .UNSPECIFIED.)
GEOMETRIC_REPRESENTATION_ITEM()
RATIONAL_B_SPLINE_SURFACE(((1.,0.705498956110755,1.),(1.,0.705821764811772,
1.),(1.,0.70646195252115,1.),(1.,0.707106781186542,1.)))
REPRESENTATION_ITEM('')
SURFACE()
);
#2902=(
BOUNDED_SURFACE()
B_SPLINE_SURFACE(3,2,((#204772,#204773,#204774),(#204775,#204776,#204777),
(#204778,#204779,#204780),(#204781,#204782,#204783)),.UNSPECIFIED.,.F.,
 .F.,.F.)
B_SPLINE_SURFACE_WITH_KNOTS((4,4),(3,3),(0.,0.00039739441082873),(0.,1.),
 .UNSPECIFIED.)
GEOMETRIC_REPRESENTATION_ITEM()
RATIONAL_B_SPLINE_SURFACE(((1.,0.708689770883327,1.),(1.,0.708376440034489,
1.),(1.,0.707750498698412,1.),(1.,0.707106781186548,1.)))
REPRESENTATION_ITEM('')
SURFACE()
);
#2903=(
BOUNDED_SURFACE()
B_SPLINE_SURFACE(3,2,((#204789,#204790,#204791),(#204792,#204793,#204794),
(#204795,#204796,#204797),(#204798,#204799,#204800)),.UNSPECIFIED.,.F.,
 .F.,.F.)
B_SPLINE_SURFACE_WITH_KNOTS((4,4),(3,3),(0.,0.000511815090126174),(0.,1.0010559227025),
 .UNSPECIFIED.)
GEOMETRIC_REPRESENTATION_ITEM()
RATIONAL_B_SPLINE_SURFACE(((1.,0.705266242717401,1.00062243213101),(1.,
0.70558408590904,1.00062176089533),(1.,0.706182089450421,1.0006204980043),
(1.,0.706797508587395,1.00061919833422)))
REPRESENTATION_ITEM('')
SURFACE()
);
#2904=(
BOUNDED_SURFACE()
B_SPLINE_SURFACE(3,2,((#204802,#204803,#204804),(#204805,#204806,#204807),
(#204808,#204809,#204810),(#204811,#204812,#204813)),.UNSPECIFIED.,.F.,
 .F.,.F.)
B_SPLINE_SURFACE_WITH_KNOTS((4,4),(3,3),(-7.58941520739853E-18,0.000397394428086626),
(0.,1.),.UNSPECIFIED.)
GEOMETRIC_REPRESENTATION_ITEM()
RATIONAL_B_SPLINE_SURFACE(((1.,0.707106781186548,1.),(1.,0.706459846759086,
1.),(1.,0.7058205107373,1.),(1.,0.705498956110753,1.)))
REPRESENTATION_ITEM('')
SURFACE()
);
#2905=(
BOUNDED_SURFACE()
B_SPLINE_SURFACE(3,2,((#204819,#204820,#204821),(#204822,#204823,#204824),
(#204825,#204826,#204827),(#204828,#204829,#204830),(#204831,#204832,#204833),
(#204834,#204835,#204836)),.UNSPECIFIED.,.F.,.F.,.F.)
B_SPLINE_SURFACE_WITH_KNOTS((4,2,4),(3,3),(0.,0.000257953807872849,0.000515907615745699),
(0.,1.),.UNSPECIFIED.)
GEOMETRIC_REPRESENTATION_ITEM()
RATIONAL_B_SPLINE_SURFACE(((1.,0.8746197071394,1.),(1.,0.874834349678804,
1.),(1.,0.854686104158048,1.),(1.,0.792476597914884,1.),(1.,0.750887854595316,
1.),(1.,0.705585838031445,1.)))
REPRESENTATION_ITEM('')
SURFACE()
);
#2906=(
BOUNDED_SURFACE()
B_SPLINE_SURFACE(3,2,((#204842,#204843,#204844),(#204845,#204846,#204847),
(#204848,#204849,#204850),(#204851,#204852,#204853)),.UNSPECIFIED.,.F.,
 .F.,.F.)
B_SPLINE_SURFACE_WITH_KNOTS((4,4),(3,3),(0.,0.000511815437699147),(0.,1.00105881331657),
 .UNSPECIFIED.)
GEOMETRIC_REPRESENTATION_ITEM()
RATIONAL_B_SPLINE_SURFACE(((1.,0.706796661946133,1.00062089519759),(1.,
0.707430821225011,1.00061955228501),(1.,0.708058545830506,1.00061822299867),
(1.,0.708394505252514,1.00061751156205)))
REPRESENTATION_ITEM('')
SURFACE()
);
#2907=(
BOUNDED_SURFACE()
B_SPLINE_SURFACE(3,2,((#204855,#204856,#204857),(#204858,#204859,#204860),
(#204861,#204862,#204863),(#204864,#204865,#204866),(#204867,#204868,#204869),
(#204870,#204871,#204872)),.UNSPECIFIED.,.F.,.F.,.F.)
B_SPLINE_SURFACE_WITH_KNOTS((4,2,4),(3,3),(0.,0.000256915317531268,0.000513830635062536),
(0.,1.),.UNSPECIFIED.)
GEOMETRIC_REPRESENTATION_ITEM()
RATIONAL_B_SPLINE_SURFACE(((1.,0.705585838031441,1.),(1.,0.750902433542207,
1.),(1.,0.792329530083274,1.),(1.,0.854288401593444,1.),(1.,0.87499803112573,
1.),(1.,0.874619707139409,1.)))
REPRESENTATION_ITEM('')
SURFACE()
);
#2908=(
BOUNDED_SURFACE()
B_SPLINE_SURFACE(3,2,((#204878,#204879,#204880),(#204881,#204882,#204883),
(#204884,#204885,#204886),(#204887,#204888,#204889),(#204890,#204891,#204892),
(#204893,#204894,#204895)),.UNSPECIFIED.,.F.,.F.,.F.)
B_SPLINE_SURFACE_WITH_KNOTS((4,2,4),(3,3),(-1.54227759036063E-17,0.000256592814262151,
0.000513185628524318),(0.,1.),.UNSPECIFIED.)
GEOMETRIC_REPRESENTATION_ITEM()
RATIONAL_B_SPLINE_SURFACE(((1.,0.708712527163657,1.),(1.,0.753780902613053,
1.),(1.,0.794538995769901,1.),(1.,0.855070770330395,1.),(1.,0.875018427445846,
1.),(1.,0.874619707139393,1.)))
REPRESENTATION_ITEM('')
SURFACE()
);
#2909=(
BOUNDED_SURFACE()
B_SPLINE_SURFACE(3,2,((#204897,#204898,#204899),(#204900,#204901,#204902),
(#204903,#204904,#204905),(#204906,#204907,#204908)),.UNSPECIFIED.,.F.,
 .F.,.F.)
B_SPLINE_SURFACE_WITH_KNOTS((4,4),(3,3),(0.,0.000511815072430394),(0.,1.00105598365931),
 .UNSPECIFIED.)
GEOMETRIC_REPRESENTATION_ITEM()
RATIONAL_B_SPLINE_SURFACE(((1.,0.706797490733558,1.00061923411731),(1.,
0.706182062146464,1.00062053388237),(1.,0.70558406276884,1.00062179683751),
(1.,0.705266224770311,1.00062246810098)))
REPRESENTATION_ITEM('')
SURFACE()
);
#2910=(
BOUNDED_SURFACE()
B_SPLINE_SURFACE(3,2,((#204914,#204915,#204916),(#204917,#204918,#204919),
(#204920,#204921,#204922),(#204923,#204924,#204925),(#204926,#204927,#204928),
(#204929,#204930,#204931)),.UNSPECIFIED.,.F.,.F.,.F.)
B_SPLINE_SURFACE_WITH_KNOTS((4,2,4),(3,3),(0.,0.000257652232350889,0.000515304464701777),
(0.,1.),.UNSPECIFIED.)
GEOMETRIC_REPRESENTATION_ITEM()
RATIONAL_B_SPLINE_SURFACE(((1.,0.874619707139377,1.),(1.,0.874861180430766,
1.),(1.,0.855455725920758,1.),(1.,0.794699358955338,1.),(1.,0.753768977788568,
1.),(1.,0.708712527163628,1.)))
REPRESENTATION_ITEM('')
SURFACE()
);
#2911=(
BOUNDED_SURFACE()
B_SPLINE_SURFACE(3,2,((#204937,#204938,#204939),(#204940,#204941,#204942),
(#204943,#204944,#204945),(#204946,#204947,#204948)),.UNSPECIFIED.,.F.,
 .F.,.F.)
B_SPLINE_SURFACE_WITH_KNOTS((4,4),(3,3),(0.,0.000397394373651908),(0.,1.),
 .UNSPECIFIED.)
GEOMETRIC_REPRESENTATION_ITEM()
RATIONAL_B_SPLINE_SURFACE(((1.,0.707106781186548,1.),(1.,0.707752587915899,
1.),(1.,0.70837765454067,1.),(1.,0.708689770883335,1.)))
REPRESENTATION_ITEM('')
SURFACE()
);
#2912=(
BOUNDED_SURFACE()
B_SPLINE_SURFACE(3,2,((#204950,#204951,#204952),(#204953,#204954,#204955),
(#204956,#204957,#204958),(#204959,#204960,#204961)),.UNSPECIFIED.,.F.,
 .F.,.F.)
B_SPLINE_SURFACE_WITH_KNOTS((4,4),(3,3),(0.,0.000511815456479795),(0.,1.00105873159874),
 .UNSPECIFIED.)
GEOMETRIC_REPRESENTATION_ITEM()
RATIONAL_B_SPLINE_SURFACE(((1.,0.708394529056711,1.00061746385291),(1.,
0.708058564167178,1.0006181752462),(1.,0.707430835372453,1.00061950443882),
(1.,0.706796685880733,1.00062084722703)))
REPRESENTATION_ITEM('')
SURFACE()
);
#2913=(
BOUNDED_SURFACE()
B_SPLINE_SURFACE(3,2,((#204967,#204968,#204969),(#204970,#204971,#204972),
(#204973,#204974,#204975),(#204976,#204977,#204978)),.UNSPECIFIED.,.F.,
 .F.,.F.)
B_SPLINE_SURFACE_WITH_KNOTS((4,4),(3,3),(0.,0.000397394465448304),(0.,1.),
 .UNSPECIFIED.)
GEOMETRIC_REPRESENTATION_ITEM()
RATIONAL_B_SPLINE_SURFACE(((1.,0.705498956110758,1.),(1.,0.705821764811759,
1.),(1.,0.706461952521154,1.),(1.,0.707106781186542,1.)))
REPRESENTATION_ITEM('')
SURFACE()
);
#2914=(
BOUNDED_SURFACE()
B_SPLINE_SURFACE(3,2,((#204984,#204985,#204986),(#204987,#204988,#204989),
(#204990,#204991,#204992),(#204993,#204994,#204995)),.UNSPECIFIED.,.F.,
 .F.,.F.)
B_SPLINE_SURFACE_WITH_KNOTS((4,4),(3,3),(0.,0.000397394410828734),(0.,1.),
 .UNSPECIFIED.)
GEOMETRIC_REPRESENTATION_ITEM()
RATIONAL_B_SPLINE_SURFACE(((1.,0.708689770883316,1.),(1.,0.708376440034496,
1.),(1.,0.707750498698412,1.),(1.,0.70710678118654,1.)))
REPRESENTATION_ITEM('')
SURFACE()
);
#2915=(
BOUNDED_SURFACE()
B_SPLINE_SURFACE(3,2,((#205001,#205002,#205003),(#205004,#205005,#205006),
(#205007,#205008,#205009),(#205010,#205011,#205012)),.UNSPECIFIED.,.F.,
 .F.,.F.)
B_SPLINE_SURFACE_WITH_KNOTS((4,4),(3,3),(0.,0.00051181509012619),(0.,1.00105592270126),
 .UNSPECIFIED.)
GEOMETRIC_REPRESENTATION_ITEM()
RATIONAL_B_SPLINE_SURFACE(((1.,0.705266242717763,1.00062243213028),(1.,
0.705584085909412,1.0006217608946),(1.,0.706182089450766,1.00062049800357),
(1.,0.706797508587757,1.0006191983335)))
REPRESENTATION_ITEM('')
SURFACE()
);
#2916=(
BOUNDED_SURFACE()
B_SPLINE_SURFACE(3,2,((#205014,#205015,#205016),(#205017,#205018,#205019),
(#205020,#205021,#205022),(#205023,#205024,#205025)),.UNSPECIFIED.,.F.,
 .F.,.F.)
B_SPLINE_SURFACE_WITH_KNOTS((4,4),(3,3),(0.,0.000397394428086627),(0.,1.),
 .UNSPECIFIED.)
GEOMETRIC_REPRESENTATION_ITEM()
RATIONAL_B_SPLINE_SURFACE(((1.,0.707106781186556,1.),(1.,0.706459846759089,
1.),(1.,0.705820510737293,1.),(1.,0.705498956110747,1.)))
REPRESENTATION_ITEM('')
SURFACE()
);
#2917=(
BOUNDED_SURFACE()
B_SPLINE_SURFACE(3,2,((#205031,#205032,#205033),(#205034,#205035,#205036),
(#205037,#205038,#205039),(#205040,#205041,#205042),(#205043,#205044,#205045),
(#205046,#205047,#205048)),.UNSPECIFIED.,.F.,.F.,.F.)
B_SPLINE_SURFACE_WITH_KNOTS((4,2,4),(3,3),(0.,0.000257953807872847,0.000515907615745694),
(0.,1.),.UNSPECIFIED.)
GEOMETRIC_REPRESENTATION_ITEM()
RATIONAL_B_SPLINE_SURFACE(((1.,0.874619707139388,1.),(1.,0.874834349679306,
1.),(1.,0.85468610415739,1.),(1.,0.792476597915524,1.),(1.,0.750887854594873,
1.),(1.,0.705585838031412,1.)))
REPRESENTATION_ITEM('')
SURFACE()
);
#2918=(
BOUNDED_SURFACE()
B_SPLINE_SURFACE(3,2,((#205054,#205055,#205056),(#205057,#205058,#205059),
(#205060,#205061,#205062),(#205063,#205064,#205065)),.UNSPECIFIED.,.F.,
 .F.,.F.)
B_SPLINE_SURFACE_WITH_KNOTS((4,4),(3,3),(0.,0.000511815437699146),(0.,1.00105881331706),
 .UNSPECIFIED.)
GEOMETRIC_REPRESENTATION_ITEM()
RATIONAL_B_SPLINE_SURFACE(((1.,0.706796661945993,1.00062089519787),(1.,
0.707430821224858,1.00061955228529),(1.,0.708058545830395,1.00061822299895),
(1.,0.708394505252372,1.00061751156233)))
REPRESENTATION_ITEM('')
SURFACE()
);
#2919=(
BOUNDED_SURFACE()
B_SPLINE_SURFACE(3,2,((#205067,#205068,#205069),(#205070,#205071,#205072),
(#205073,#205074,#205075),(#205076,#205077,#205078),(#205079,#205080,#205081),
(#205082,#205083,#205084)),.UNSPECIFIED.,.F.,.F.,.F.)
B_SPLINE_SURFACE_WITH_KNOTS((4,2,4),(3,3),(0.,0.000256915317531268,0.000513830635062537),
(0.,1.),.UNSPECIFIED.)
GEOMETRIC_REPRESENTATION_ITEM()
RATIONAL_B_SPLINE_SURFACE(((1.,0.705585838031444,1.),(1.,0.750902433542666,
1.),(1.,0.792329530082642,1.),(1.,0.854288401594098,1.),(1.,0.874998031125232,
1.),(1.,0.874619707139418,1.)))
REPRESENTATION_ITEM('')
SURFACE()
);
#2920=(
BOUNDED_SURFACE()
B_SPLINE_SURFACE(3,2,((#205090,#205091,#205092),(#205093,#205094,#205095),
(#205096,#205097,#205098),(#205099,#205100,#205101),(#205102,#205103,#205104),
(#205105,#205106,#205107)),.UNSPECIFIED.,.F.,.F.,.F.)
B_SPLINE_SURFACE_WITH_KNOTS((4,2,4),(3,3),(-9.59518922649671E-18,0.000256592814262151,
0.000513185628524311),(0.,1.),.UNSPECIFIED.)
GEOMETRIC_REPRESENTATION_ITEM()
RATIONAL_B_SPLINE_SURFACE(((1.,0.70871252716365,1.),(1.,0.753780902613946,
1.),(1.,0.794538995768726,1.),(1.,0.855070770331594,1.),(1.,0.875018427444952,
1.),(1.,0.874619707139389,1.)))
REPRESENTATION_ITEM('')
SURFACE()
);
#2921=(
BOUNDED_SURFACE()
B_SPLINE_SURFACE(3,2,((#205109,#205110,#205111),(#205112,#205113,#205114),
(#205115,#205116,#205117),(#205118,#205119,#205120)),.UNSPECIFIED.,.F.,
 .F.,.F.)
B_SPLINE_SURFACE_WITH_KNOTS((4,4),(3,3),(0.,0.000511815072430389),(0.,1.00105598365899),
 .UNSPECIFIED.)
GEOMETRIC_REPRESENTATION_ITEM()
RATIONAL_B_SPLINE_SURFACE(((1.,0.706797490733651,1.00061923411712),(1.,
0.706182062146583,1.00062053388218),(1.,0.705584062768932,1.00062179683732),
(1.,0.705266224770413,1.00062246810079)))
REPRESENTATION_ITEM('')
SURFACE()
);
#2922=(
BOUNDED_SURFACE()
B_SPLINE_SURFACE(3,2,((#205126,#205127,#205128),(#205129,#205130,#205131),
(#205132,#205133,#205134),(#205135,#205136,#205137),(#205138,#205139,#205140),
(#205141,#205142,#205143)),.UNSPECIFIED.,.F.,.F.,.F.)
B_SPLINE_SURFACE_WITH_KNOTS((4,2,4),(3,3),(-1.35525271560688E-20,0.000257652232350883,
0.000515304464701766),(0.,1.),.UNSPECIFIED.)
GEOMETRIC_REPRESENTATION_ITEM()
RATIONAL_B_SPLINE_SURFACE(((1.,0.874619707139374,1.),(1.,0.874861180430592,
1.),(1.,0.855455725921011,1.),(1.,0.794699358955083,1.),(1.,0.753768977788722,
1.),(1.,0.708712527163651,1.)))
REPRESENTATION_ITEM('')
SURFACE()
);
#2923=(
BOUNDED_SURFACE()
B_SPLINE_SURFACE(3,2,((#205149,#205150,#205151),(#205152,#205153,#205154),
(#205155,#205156,#205157),(#205158,#205159,#205160)),.UNSPECIFIED.,.F.,
 .F.,.F.)
B_SPLINE_SURFACE_WITH_KNOTS((4,4),(3,3),(-1.52601455777335E-17,0.000397394373651901),
(0.,1.),.UNSPECIFIED.)
GEOMETRIC_REPRESENTATION_ITEM()
RATIONAL_B_SPLINE_SURFACE(((1.,0.707106781186547,1.),(1.,0.707752587915871,
1.),(1.,0.708377654540695,1.),(1.,0.708689770883342,1.)))
REPRESENTATION_ITEM('')
SURFACE()
);
#2924=(
BOUNDED_SURFACE()
B_SPLINE_SURFACE(3,2,((#205162,#205163,#205164),(#205165,#205166,#205167),
(#205168,#205169,#205170),(#205171,#205172,#205173)),.UNSPECIFIED.,.F.,
 .F.,.F.)
B_SPLINE_SURFACE_WITH_KNOTS((4,4),(3,3),(0.,0.000511815456479782),(0.,1.00105873159867),
 .UNSPECIFIED.)
GEOMETRIC_REPRESENTATION_ITEM()
RATIONAL_B_SPLINE_SURFACE(((1.,0.708394529056701,1.00061746385287),(1.,
0.708058564167264,1.00061817524616),(1.,0.707430835372431,1.00061950443878),
(1.,0.706796685880745,1.00062084722699)))
REPRESENTATION_ITEM('')
SURFACE()
);
#2925=(
BOUNDED_SURFACE()
B_SPLINE_SURFACE(3,2,((#205179,#205180,#205181),(#205182,#205183,#205184),
(#205185,#205186,#205187),(#205188,#205189,#205190)),.UNSPECIFIED.,.F.,
 .F.,.F.)
B_SPLINE_SURFACE_WITH_KNOTS((4,4),(3,3),(0.,0.000397394465448317),(0.,1.),
 .UNSPECIFIED.)
GEOMETRIC_REPRESENTATION_ITEM()
RATIONAL_B_SPLINE_SURFACE(((1.,0.705498956110763,1.),(1.,0.705821764811761,
1.),(1.,0.706461952521164,1.),(1.,0.707106781186548,1.)))
REPRESENTATION_ITEM('')
SURFACE()
);
#2926=(
BOUNDED_SURFACE()
B_SPLINE_SURFACE(3,2,((#205196,#205197,#205198),(#205199,#205200,#205201),
(#205202,#205203,#205204),(#205205,#205206,#205207)),.UNSPECIFIED.,.F.,
 .F.,.F.)
B_SPLINE_SURFACE_WITH_KNOTS((4,4),(3,3),(0.,0.000397394410828733),(0.,1.),
 .UNSPECIFIED.)
GEOMETRIC_REPRESENTATION_ITEM()
RATIONAL_B_SPLINE_SURFACE(((1.,0.708689770883334,1.),(1.,0.708376440034487,
1.),(1.,0.707750498698412,1.),(1.,0.707106781186548,1.)))
REPRESENTATION_ITEM('')
SURFACE()
);
#2927=(
BOUNDED_SURFACE()
B_SPLINE_SURFACE(3,2,((#205213,#205214,#205215),(#205216,#205217,#205218),
(#205219,#205220,#205221),(#205222,#205223,#205224)),.UNSPECIFIED.,.F.,
 .F.,.F.)
B_SPLINE_SURFACE_WITH_KNOTS((4,4),(3,3),(0.,0.000511815090126187),(0.,1.00105592270036),
 .UNSPECIFIED.)
GEOMETRIC_REPRESENTATION_ITEM()
RATIONAL_B_SPLINE_SURFACE(((1.,0.705266242718023,1.00062243212976),(1.,
0.705584085909673,1.00062176089407),(1.,0.706182089451057,1.00062049800304),
(1.,0.70679750858802,1.00061919833297)))
REPRESENTATION_ITEM('')
SURFACE()
);
#2928=(
BOUNDED_SURFACE()
B_SPLINE_SURFACE(3,2,((#205226,#205227,#205228),(#205229,#205230,#205231),
(#205232,#205233,#205234),(#205235,#205236,#205237)),.UNSPECIFIED.,.F.,
 .F.,.F.)
B_SPLINE_SURFACE_WITH_KNOTS((4,4),(3,3),(0.,0.000397394428086623),(0.,1.),
 .UNSPECIFIED.)
GEOMETRIC_REPRESENTATION_ITEM()
RATIONAL_B_SPLINE_SURFACE(((1.,0.707106781186548,1.),(1.,0.706459846759091,
1.),(1.,0.705820510737279,1.),(1.,0.705498956110749,1.)))
REPRESENTATION_ITEM('')
SURFACE()
);
#2929=(
BOUNDED_SURFACE()
B_SPLINE_SURFACE(3,2,((#205243,#205244,#205245),(#205246,#205247,#205248),
(#205249,#205250,#205251),(#205252,#205253,#205254),(#205255,#205256,#205257),
(#205258,#205259,#205260)),.UNSPECIFIED.,.F.,.F.,.F.)
B_SPLINE_SURFACE_WITH_KNOTS((4,2,4),(3,3),(0.,0.000257953807872846,0.000515907615745693),
(0.,1.),.UNSPECIFIED.)
GEOMETRIC_REPRESENTATION_ITEM()
RATIONAL_B_SPLINE_SURFACE(((1.,0.874619707139391,1.),(1.,0.874834349679337,
1.),(1.,0.854686104157324,1.),(1.,0.792476597915613,1.),(1.,0.750887854594759,
1.),(1.,0.705585838031461,1.)))
REPRESENTATION_ITEM('')
SURFACE()
);
#2930=(
BOUNDED_SURFACE()
B_SPLINE_SURFACE(3,2,((#205266,#205267,#205268),(#205269,#205270,#205271),
(#205272,#205273,#205274),(#205275,#205276,#205277)),.UNSPECIFIED.,.F.,
 .F.,.F.)
B_SPLINE_SURFACE_WITH_KNOTS((4,4),(3,3),(0.,0.000511815437699162),(0.,1.00105881331649),
 .UNSPECIFIED.)
GEOMETRIC_REPRESENTATION_ITEM()
RATIONAL_B_SPLINE_SURFACE(((1.,0.706796661946159,1.00062089519754),(1.,
0.707430821225023,1.00061955228496),(1.,0.708058545830554,1.00061822299862),
(1.,0.708394505252524,1.000617511562)))
REPRESENTATION_ITEM('')
SURFACE()
);
#2931=(
BOUNDED_SURFACE()
B_SPLINE_SURFACE(3,2,((#205279,#205280,#205281),(#205282,#205283,#205284),
(#205285,#205286,#205287),(#205288,#205289,#205290),(#205291,#205292,#205293),
(#205294,#205295,#205296)),.UNSPECIFIED.,.F.,.F.,.F.)
B_SPLINE_SURFACE_WITH_KNOTS((4,2,4),(3,3),(0.,0.000256915317531264,0.000513830635062528),
(0.,1.),.UNSPECIFIED.)
GEOMETRIC_REPRESENTATION_ITEM()
RATIONAL_B_SPLINE_SURFACE(((1.,0.705585838031427,1.),(1.,0.750902433542537,
1.),(1.,0.792329530082828,1.),(1.,0.854288401593886,1.),(1.,0.874998031125381,
1.),(1.,0.874619707139383,1.)))
REPRESENTATION_ITEM('')
SURFACE()
);
#2932=(
BOUNDED_SURFACE()
B_SPLINE_SURFACE(3,2,((#205302,#205303,#205304),(#205305,#205306,#205307),
(#205308,#205309,#205310),(#205311,#205312,#205313),(#205314,#205315,#205316),
(#205317,#205318,#205319)),.UNSPECIFIED.,.F.,.F.,.F.)
B_SPLINE_SURFACE_WITH_KNOTS((4,2,4),(3,3),(-5.77337656848531E-18,0.000256592814262161,
0.000513185628524327),(0.,1.),.UNSPECIFIED.)
GEOMETRIC_REPRESENTATION_ITEM()
RATIONAL_B_SPLINE_SURFACE(((1.,0.708712527163664,1.),(1.,0.753780902613862,
1.),(1.,0.79453899576885,1.),(1.,0.855070770331452,1.),(1.,0.875018427445077,
1.),(1.,0.874619707139383,1.)))
REPRESENTATION_ITEM('')
SURFACE()
);
#2933=(
BOUNDED_SURFACE()
B_SPLINE_SURFACE(3,2,((#205321,#205322,#205323),(#205324,#205325,#205326),
(#205327,#205328,#205329),(#205330,#205331,#205332)),.UNSPECIFIED.,.F.,
 .F.,.F.)
B_SPLINE_SURFACE_WITH_KNOTS((4,4),(3,3),(0.,0.000511815072430397),(0.,1.00105598365653),
 .UNSPECIFIED.)
GEOMETRIC_REPRESENTATION_ITEM()
RATIONAL_B_SPLINE_SURFACE(((1.,0.706797490734371,1.00061923411568),(1.,
0.706182062147292,1.00062053388074),(1.,0.705584062769647,1.00062179683588),
(1.,0.705266224771127,1.00062246809934)))
REPRESENTATION_ITEM('')
SURFACE()
);
#2934=(
BOUNDED_SURFACE()
B_SPLINE_SURFACE(3,2,((#205338,#205339,#205340),(#205341,#205342,#205343),
(#205344,#205345,#205346),(#205347,#205348,#205349),(#205350,#205351,#205352),
(#205353,#205354,#205355)),.UNSPECIFIED.,.F.,.F.,.F.)
B_SPLINE_SURFACE_WITH_KNOTS((4,2,4),(3,3),(0.,0.000257652232350883,0.000515304464701766),
(0.,1.),.UNSPECIFIED.)
GEOMETRIC_REPRESENTATION_ITEM()
RATIONAL_B_SPLINE_SURFACE(((1.,0.874619707139394,1.),(1.,0.874861180431301,
1.),(1.,0.855455725920046,1.),(1.,0.794699358956096,1.),(1.,0.753768977788045,
1.),(1.,0.708712527163649,1.)))
REPRESENTATION_ITEM('')
SURFACE()
);
#2935=(
BOUNDED_SURFACE()
B_SPLINE_SURFACE(3,2,((#205361,#205362,#205363),(#205364,#205365,#205366),
(#205367,#205368,#205369),(#205370,#205371,#205372)),.UNSPECIFIED.,.F.,
 .F.,.F.)
B_SPLINE_SURFACE_WITH_KNOTS((4,4),(3,3),(0.,0.000397394373651916),(0.,1.),
 .UNSPECIFIED.)
GEOMETRIC_REPRESENTATION_ITEM()
RATIONAL_B_SPLINE_SURFACE(((1.,0.707106781186546,1.),(1.,0.707752587915909,
1.),(1.,0.708377654540654,1.),(1.,0.708689770883326,1.)))
REPRESENTATION_ITEM('')
SURFACE()
);
#2936=(
BOUNDED_SURFACE()
B_SPLINE_SURFACE(3,2,((#205374,#205375,#205376),(#205377,#205378,#205379),
(#205380,#205381,#205382),(#205383,#205384,#205385)),.UNSPECIFIED.,.F.,
 .F.,.F.)
B_SPLINE_SURFACE_WITH_KNOTS((4,4),(3,3),(0.,0.000511815456479791),(0.,1.00105873159914),
 .UNSPECIFIED.)
GEOMETRIC_REPRESENTATION_ITEM()
RATIONAL_B_SPLINE_SURFACE(((1.,0.708394529056566,1.00061746385314),(1.,
0.708058564167089,1.00061817524643),(1.,0.707430835372312,1.00061950443905),
(1.,0.706796685880615,1.00062084722726)))
REPRESENTATION_ITEM('')
SURFACE()
);
#2937=(
BOUNDED_SURFACE()
B_SPLINE_SURFACE(3,2,((#205391,#205392,#205393),(#205394,#205395,#205396),
(#205397,#205398,#205399),(#205400,#205401,#205402)),.UNSPECIFIED.,.F.,
 .F.,.F.)
B_SPLINE_SURFACE_WITH_KNOTS((4,4),(3,3),(0.,0.000397394465448314),(0.,1.),
 .UNSPECIFIED.)
GEOMETRIC_REPRESENTATION_ITEM()
RATIONAL_B_SPLINE_SURFACE(((1.,0.705498956110748,1.),(1.,0.705821764811775,
1.),(1.,0.706461952521155,1.),(1.,0.707106781186531,1.)))
REPRESENTATION_ITEM('')
SURFACE()
);
#2938=(
BOUNDED_SURFACE()
B_SPLINE_SURFACE(3,2,((#205408,#205409,#205410),(#205411,#205412,#205413),
(#205414,#205415,#205416),(#205417,#205418,#205419)),.UNSPECIFIED.,.F.,
 .F.,.F.)
B_SPLINE_SURFACE_WITH_KNOTS((4,4),(3,3),(0.,0.000397394410828728),(0.,1.),
 .UNSPECIFIED.)
GEOMETRIC_REPRESENTATION_ITEM()
RATIONAL_B_SPLINE_SURFACE(((1.,0.708689770883322,1.),(1.,0.708376440034482,
1.),(1.,0.707750498698425,1.),(1.,0.707106781186525,1.)))
REPRESENTATION_ITEM('')
SURFACE()
);
#2939=(
BOUNDED_SURFACE()
B_SPLINE_SURFACE(3,2,((#205425,#205426,#205427),(#205428,#205429,#205430),
(#205431,#205432,#205433),(#205434,#205435,#205436)),.UNSPECIFIED.,.F.,
 .F.,.F.)
B_SPLINE_SURFACE_WITH_KNOTS((4,4),(3,3),(0.,0.000511815090126179),(0.,1.00105592269913),
 .UNSPECIFIED.)
GEOMETRIC_REPRESENTATION_ITEM()
RATIONAL_B_SPLINE_SURFACE(((1.,0.705266242718401,1.00062243212903),(1.,
0.705584085910067,1.00062176089334),(1.,0.706182089451372,1.00062049800232),
(1.,0.706797508588382,1.00061919833224)))
REPRESENTATION_ITEM('')
SURFACE()
);
#2940=(
BOUNDED_SURFACE()
B_SPLINE_SURFACE(3,2,((#205438,#205439,#205440),(#205441,#205442,#205443),
(#205444,#205445,#205446),(#205447,#205448,#205449)),.UNSPECIFIED.,.F.,
 .F.,.F.)
B_SPLINE_SURFACE_WITH_KNOTS((4,4),(3,3),(0.,0.000397394428086626),(0.,1.),
 .UNSPECIFIED.)
GEOMETRIC_REPRESENTATION_ITEM()
RATIONAL_B_SPLINE_SURFACE(((1.,0.707106781186536,1.),(1.,0.706459846759119,
1.),(1.,0.705820510737292,1.),(1.,0.705498956110736,1.)))
REPRESENTATION_ITEM('')
SURFACE()
);
#2941=(
BOUNDED_SURFACE()
B_SPLINE_SURFACE(3,2,((#205455,#205456,#205457),(#205458,#205459,#205460),
(#205461,#205462,#205463),(#205464,#205465,#205466),(#205467,#205468,#205469),
(#205470,#205471,#205472)),.UNSPECIFIED.,.F.,.F.,.F.)
B_SPLINE_SURFACE_WITH_KNOTS((4,2,4),(3,3),(0.,0.000257953807872847,0.000515907615745694),
(0.,1.),.UNSPECIFIED.)
GEOMETRIC_REPRESENTATION_ITEM()
RATIONAL_B_SPLINE_SURFACE(((1.,0.874619707139395,1.),(1.,0.874834349679049,
1.),(1.,0.854686104157715,1.),(1.,0.792476597915225,1.),(1.,0.750887854595061,
1.),(1.,0.705585838031448,1.)))
REPRESENTATION_ITEM('')
SURFACE()
);
#2942=(
BOUNDED_SURFACE()
B_SPLINE_SURFACE(3,2,((#205478,#205479,#205480),(#205481,#205482,#205483),
(#205484,#205485,#205486),(#205487,#205488,#205489)),.UNSPECIFIED.,.F.,
 .F.,.F.)
B_SPLINE_SURFACE_WITH_KNOTS((4,4),(3,3),(0.,0.00051181543769915),(0.,1.00105881331433),
 .UNSPECIFIED.)
GEOMETRIC_REPRESENTATION_ITEM()
RATIONAL_B_SPLINE_SURFACE(((1.,0.706796661946792,1.00062089519627),(1.,
0.707430821225683,1.0006195522837),(1.,0.708058545831151,1.00061822299736),
(1.,0.708394505253171,1.00061751156074)))
REPRESENTATION_ITEM('')
SURFACE()
);
#2943=(
BOUNDED_SURFACE()
B_SPLINE_SURFACE(3,2,((#205491,#205492,#205493),(#205494,#205495,#205496),
(#205497,#205498,#205499),(#205500,#205501,#205502),(#205503,#205504,#205505),
(#205506,#205507,#205508)),.UNSPECIFIED.,.F.,.F.,.F.)
B_SPLINE_SURFACE_WITH_KNOTS((4,2,4),(3,3),(0.,0.000256915317531265,0.00051383063506253),
(0.,1.),.UNSPECIFIED.)
GEOMETRIC_REPRESENTATION_ITEM()
RATIONAL_B_SPLINE_SURFACE(((1.,0.705585838031436,1.),(1.,0.7509024335433,
1.),(1.,0.792329530081799,1.),(1.,0.854288401594921,1.),(1.,0.874998031124604,
1.),(1.,0.874619707139392,1.)))
REPRESENTATION_ITEM('')
SURFACE()
);
#2944=(
BOUNDED_SURFACE()
B_SPLINE_SURFACE(3,2,((#205514,#205515,#205516),(#205517,#205518,#205519),
(#205520,#205521,#205522),(#205523,#205524,#205525),(#205526,#205527,#205528),
(#205529,#205530,#205531)),.UNSPECIFIED.,.F.,.F.,.F.)
B_SPLINE_SURFACE_WITH_KNOTS((4,2,4),(3,3),(0.,0.000256592814262157,0.000513185628524315),
(0.,1.),.UNSPECIFIED.)
GEOMETRIC_REPRESENTATION_ITEM()
RATIONAL_B_SPLINE_SURFACE(((1.,0.708712527163664,1.),(1.,0.753780902613349,
1.),(1.,0.794538995769515,1.),(1.,0.855070770330789,1.),(1.,0.875018427445547,
1.),(1.,0.874619707139392,1.)))
REPRESENTATION_ITEM('')
SURFACE()
);
#2945=(
BOUNDED_SURFACE()
B_SPLINE_SURFACE(3,2,((#205533,#205534,#205535),(#205536,#205537,#205538),
(#205539,#205540,#205541),(#205542,#205543,#205544)),.UNSPECIFIED.,.F.,
 .F.,.F.)
B_SPLINE_SURFACE_WITH_KNOTS((4,4),(3,3),(0.,0.000511815072430392),(0.,1.00105598365706),
 .UNSPECIFIED.)
GEOMETRIC_REPRESENTATION_ITEM()
RATIONAL_B_SPLINE_SURFACE(((1.,0.706797490734217,1.00061923411599),(1.,
0.706182062147139,1.00062053388105),(1.,0.705584062769492,1.00062179683619),
(1.,0.705266224770975,1.00062246809965)))
REPRESENTATION_ITEM('')
SURFACE()
);
#2946=(
BOUNDED_SURFACE()
B_SPLINE_SURFACE(3,2,((#205550,#205551,#205552),(#205553,#205554,#205555),
(#205556,#205557,#205558),(#205559,#205560,#205561),(#205562,#205563,#205564),
(#205565,#205566,#205567)),.UNSPECIFIED.,.F.,.F.,.F.)
B_SPLINE_SURFACE_WITH_KNOTS((4,2,4),(3,3),(0.,0.000257652232350882,0.000515304464701764),
(0.,1.),.UNSPECIFIED.)
GEOMETRIC_REPRESENTATION_ITEM()
RATIONAL_B_SPLINE_SURFACE(((1.,0.874619707139393,1.),(1.,0.874861180431177,
1.),(1.,0.855455725920209,1.),(1.,0.794699358955939,1.),(1.,0.7537689777881,
1.),(1.,0.70871252716366,1.)))
REPRESENTATION_ITEM('')
SURFACE()
);
#2947=(
BOUNDED_SURFACE()
B_SPLINE_SURFACE(3,2,((#205573,#205574,#205575),(#205576,#205577,#205578),
(#205579,#205580,#205581),(#205582,#205583,#205584)),.UNSPECIFIED.,.F.,
 .F.,.F.)
B_SPLINE_SURFACE_WITH_KNOTS((4,4),(3,3),(-9.56808417218458E-18,0.000397394373651918),
(0.,1.),.UNSPECIFIED.)
GEOMETRIC_REPRESENTATION_ITEM()
RATIONAL_B_SPLINE_SURFACE(((1.,0.707106781186559,1.),(1.,0.707752587915889,
1.),(1.,0.708377654540676,1.),(1.,0.708689770883342,1.)))
REPRESENTATION_ITEM('')
SURFACE()
);
#2948=(
BOUNDED_SURFACE()
B_SPLINE_SURFACE(3,2,((#205586,#205587,#205588),(#205589,#205590,#205591),
(#205592,#205593,#205594),(#205595,#205596,#205597)),.UNSPECIFIED.,.F.,
 .F.,.F.)
B_SPLINE_SURFACE_WITH_KNOTS((4,4),(3,3),(0.,0.000511815456479788),(0.,1.00105873160029),
 .UNSPECIFIED.)
GEOMETRIC_REPRESENTATION_ITEM()
RATIONAL_B_SPLINE_SURFACE(((1.,0.70839452905621,1.00061746385381),(1.,0.708058564166803,
1.0006181752471),(1.,0.707430835371955,1.00061950443973),(1.,0.706796685880289,
1.00062084722794)))
REPRESENTATION_ITEM('')
SURFACE()
);
#2949=(
BOUNDED_SURFACE()
B_SPLINE_SURFACE(3,2,((#205603,#205604,#205605),(#205606,#205607,#205608),
(#205609,#205610,#205611),(#205612,#205613,#205614)),.UNSPECIFIED.,.F.,
 .F.,.F.)
B_SPLINE_SURFACE_WITH_KNOTS((4,4),(3,3),(-6.53231808922516E-18,0.000397394465448321),
(0.,1.),.UNSPECIFIED.)
GEOMETRIC_REPRESENTATION_ITEM()
RATIONAL_B_SPLINE_SURFACE(((1.,0.705498956110736,1.),(1.,0.705821764811783,
1.),(1.,0.706461952521136,1.),(1.,0.707106781186559,1.)))
REPRESENTATION_ITEM('')
SURFACE()
);
#2950=(
BOUNDED_SURFACE()
B_SPLINE_SURFACE(3,2,((#205620,#205621,#205622),(#205623,#205624,#205625),
(#205626,#205627,#205628),(#205629,#205630,#205631)),.UNSPECIFIED.,.F.,
 .F.,.F.)
B_SPLINE_SURFACE_WITH_KNOTS((4,4),(3,3),(0.,0.000397394410828731),(0.,1.),
 .UNSPECIFIED.)
GEOMETRIC_REPRESENTATION_ITEM()
RATIONAL_B_SPLINE_SURFACE(((1.,0.708689770883326,1.),(1.,0.708376440034496,
1.),(1.,0.707750498698427,1.),(1.,0.707106781186548,1.)))
REPRESENTATION_ITEM('')
SURFACE()
);
#2951=(
BOUNDED_SURFACE()
B_SPLINE_SURFACE(3,2,((#205637,#205638,#205639),(#205640,#205641,#205642),
(#205643,#205644,#205645),(#205646,#205647,#205648)),.UNSPECIFIED.,.F.,
 .F.,.F.)
B_SPLINE_SURFACE_WITH_KNOTS((4,4),(3,3),(0.,0.000511815090126171),(0.,1.0010559227001),
 .UNSPECIFIED.)
GEOMETRIC_REPRESENTATION_ITEM()
RATIONAL_B_SPLINE_SURFACE(((1.,0.705266242718086,1.0006224321296),(1.,0.705584085909776,
1.00062176089391),(1.,0.706182089451097,1.00062049800289),(1.,0.706797508588098,
1.00061919833281)))
REPRESENTATION_ITEM('')
SURFACE()
);
#2952=(
BOUNDED_SURFACE()
B_SPLINE_SURFACE(3,2,((#205650,#205651,#205652),(#205653,#205654,#205655),
(#205656,#205657,#205658),(#205659,#205660,#205661)),.UNSPECIFIED.,.F.,
 .F.,.F.)
B_SPLINE_SURFACE_WITH_KNOTS((4,4),(3,3),(0.,0.000397394428086631),(0.,1.),
 .UNSPECIFIED.)
GEOMETRIC_REPRESENTATION_ITEM()
RATIONAL_B_SPLINE_SURFACE(((1.,0.707106781186548,1.),(1.,0.706459846759102,
1.),(1.,0.70582051073727,1.),(1.,0.705498956110742,1.)))
REPRESENTATION_ITEM('')
SURFACE()
);
#2953=(
BOUNDED_SURFACE()
B_SPLINE_SURFACE(3,2,((#205667,#205668,#205669),(#205670,#205671,#205672),
(#205673,#205674,#205675),(#205676,#205677,#205678),(#205679,#205680,#205681),
(#205682,#205683,#205684)),.UNSPECIFIED.,.F.,.F.,.F.)
B_SPLINE_SURFACE_WITH_KNOTS((4,2,4),(3,3),(0.,0.000257953807872848,0.000515907615745695),
(0.,1.),.UNSPECIFIED.)
GEOMETRIC_REPRESENTATION_ITEM()
RATIONAL_B_SPLINE_SURFACE(((1.,0.874619707139383,1.),(1.,0.874834349678855,
1.),(1.,0.854686104157979,1.),(1.,0.79247659791496,1.),(1.,0.750887854595262,
1.),(1.,0.705585838031416,1.)))
REPRESENTATION_ITEM('')
SURFACE()
);
#2954=(
BOUNDED_SURFACE()
B_SPLINE_SURFACE(3,2,((#205690,#205691,#205692),(#205693,#205694,#205695),
(#205696,#205697,#205698),(#205699,#205700,#205701)),.UNSPECIFIED.,.F.,
 .F.,.F.)
B_SPLINE_SURFACE_WITH_KNOTS((4,4),(3,3),(0.,0.000511815437699153),(0.,1.00105881331625),
 .UNSPECIFIED.)
GEOMETRIC_REPRESENTATION_ITEM()
RATIONAL_B_SPLINE_SURFACE(((1.,0.706796661946227,1.0006208951974),(1.,0.707430821225108,
1.00061955228482),(1.,0.708058545830617,1.00061822299848),(1.,0.708394505252617,
1.00061751156186)))
REPRESENTATION_ITEM('')
SURFACE()
);
#2955=(
BOUNDED_SURFACE()
B_SPLINE_SURFACE(3,2,((#205703,#205704,#205705),(#205706,#205707,#205708),
(#205709,#205710,#205711),(#205712,#205713,#205714),(#205715,#205716,#205717),
(#205718,#205719,#205720)),.UNSPECIFIED.,.F.,.F.,.F.)
B_SPLINE_SURFACE_WITH_KNOTS((4,2,4),(3,3),(-9.37834879199961E-18,0.000256915317531254,
0.000513830635062517),(0.,1.),.UNSPECIFIED.)
GEOMETRIC_REPRESENTATION_ITEM()
RATIONAL_B_SPLINE_SURFACE(((1.,0.705585838031447,1.),(1.,0.750902433543063,
1.),(1.,0.79232953008209,1.),(1.,0.854288401594609,1.),(1.,0.874998031124818,
1.),(1.,0.87461970713939,1.)))
REPRESENTATION_ITEM('')
SURFACE()
);
#2956=(
BOUNDED_SURFACE()
B_SPLINE_SURFACE(3,2,((#205726,#205727,#205728),(#205729,#205730,#205731),
(#205732,#205733,#205734),(#205735,#205736,#205737),(#205738,#205739,#205740),
(#205741,#205742,#205743)),.UNSPECIFIED.,.F.,.F.,.F.)
B_SPLINE_SURFACE_WITH_KNOTS((4,2,4),(3,3),(-9.32413868337534E-18,0.000256592814262153,
0.000513185628524315),(0.,1.),.UNSPECIFIED.)
GEOMETRIC_REPRESENTATION_ITEM()
RATIONAL_B_SPLINE_SURFACE(((1.,0.708712527163675,1.),(1.,0.753780902613636,
1.),(1.,0.794538995769133,1.),(1.,0.855070770331152,1.),(1.,0.875018427445287,
1.),(1.,0.874619707139396,1.)))
REPRESENTATION_ITEM('')
SURFACE()
);
#2957=(
BOUNDED_SURFACE()
B_SPLINE_SURFACE(3,2,((#205745,#205746,#205747),(#205748,#205749,#205750),
(#205751,#205752,#205753),(#205754,#205755,#205756)),.UNSPECIFIED.,.F.,
 .F.,.F.)
B_SPLINE_SURFACE_WITH_KNOTS((4,4),(3,3),(0.,0.000511815072430401),(0.,1.00105598365716),
 .UNSPECIFIED.)
GEOMETRIC_REPRESENTATION_ITEM()
RATIONAL_B_SPLINE_SURFACE(((1.,0.706797490734188,1.00061923411604),(1.,
0.706182062147101,1.0006205338811),(1.,0.705584062769487,1.00062179683624),
(1.,0.705266224770961,1.00062246809971)))
REPRESENTATION_ITEM('')
SURFACE()
);
#2958=(
BOUNDED_SURFACE()
B_SPLINE_SURFACE(3,2,((#205762,#205763,#205764),(#205765,#205766,#205767),
(#205768,#205769,#205770),(#205771,#205772,#205773),(#205774,#205775,#205776),
(#205777,#205778,#205779)),.UNSPECIFIED.,.F.,.F.,.F.)
B_SPLINE_SURFACE_WITH_KNOTS((4,2,4),(3,3),(-9.62229428080885E-18,0.000257652232350869,
0.000515304464701747),(0.,1.),.UNSPECIFIED.)
GEOMETRIC_REPRESENTATION_ITEM()
RATIONAL_B_SPLINE_SURFACE(((1.,0.874619707139388,1.),(1.,0.87486118043047,
1.),(1.,0.855455725921216,1.),(1.,0.794699358954906,1.),(1.,0.753768977788931,
1.),(1.,0.70871252716366,1.)))
REPRESENTATION_ITEM('')
SURFACE()
);
#2959=(
BOUNDED_SURFACE()
B_SPLINE_SURFACE(3,2,((#205785,#205786,#205787),(#205788,#205789,#205790),
(#205791,#205792,#205793),(#205794,#205795,#205796)),.UNSPECIFIED.,.F.,
 .F.,.F.)
B_SPLINE_SURFACE_WITH_KNOTS((4,4),(3,3),(0.,0.000397394373651925),(0.,1.),
 .UNSPECIFIED.)
GEOMETRIC_REPRESENTATION_ITEM()
RATIONAL_B_SPLINE_SURFACE(((1.,0.707106781186548,1.),(1.,0.707752587915922,
1.),(1.,0.708377654540667,1.),(1.,0.708689770883311,1.)))
REPRESENTATION_ITEM('')
SURFACE()
);
#2960=(
BOUNDED_SURFACE()
B_SPLINE_SURFACE(3,2,((#205798,#205799,#205800),(#205801,#205802,#205803),
(#205804,#205805,#205806),(#205807,#205808,#205809)),.UNSPECIFIED.,.F.,
 .F.,.F.)
B_SPLINE_SURFACE_WITH_KNOTS((4,4),(3,3),(0.,0.000511815456479788),(0.,1.0010587316027),
 .UNSPECIFIED.)
GEOMETRIC_REPRESENTATION_ITEM()
RATIONAL_B_SPLINE_SURFACE(((1.,0.708394529055522,1.00061746385522),(1.,
0.7080585641661,1.00061817524851),(1.,0.70743083537124,1.00061950444114),
(1.,0.706796685879573,1.00062084722935)))
REPRESENTATION_ITEM('')
SURFACE()
);
#2961=(
BOUNDED_SURFACE()
B_SPLINE_SURFACE(3,2,((#205815,#205816,#205817),(#205818,#205819,#205820),
(#205821,#205822,#205823),(#205824,#205825,#205826)),.UNSPECIFIED.,.F.,
 .F.,.F.)
B_SPLINE_SURFACE_WITH_KNOTS((4,4),(3,3),(0.,0.000397394465448303),(0.,1.),
 .UNSPECIFIED.)
GEOMETRIC_REPRESENTATION_ITEM()
RATIONAL_B_SPLINE_SURFACE(((1.,0.705498956110765,1.),(1.,0.705821764811767,
1.),(1.,0.706461952521164,1.),(1.,0.707106781186548,1.)))
REPRESENTATION_ITEM('')
SURFACE()
);
#2962=(
BOUNDED_SURFACE()
B_SPLINE_SURFACE(3,2,((#205832,#205833,#205834),(#205835,#205836,#205837),
(#205838,#205839,#205840),(#205841,#205842,#205843)),.UNSPECIFIED.,.F.,
 .F.,.F.)
B_SPLINE_SURFACE_WITH_KNOTS((4,4),(3,3),(0.,0.000397394410828739),(0.,1.),
 .UNSPECIFIED.)
GEOMETRIC_REPRESENTATION_ITEM()
RATIONAL_B_SPLINE_SURFACE(((1.,0.708689770883324,1.),(1.,0.708376440034488,
1.),(1.,0.707750498698415,1.),(1.,0.707106781186548,1.)))
REPRESENTATION_ITEM('')
SURFACE()
);
#2963=(
BOUNDED_SURFACE()
B_SPLINE_SURFACE(3,2,((#205849,#205850,#205851),(#205852,#205853,#205854),
(#205855,#205856,#205857),(#205858,#205859,#205860)),.UNSPECIFIED.,.F.,
 .F.,.F.)
B_SPLINE_SURFACE_WITH_KNOTS((4,4),(3,3),(0.,0.000511815090126181),(0.,1.00105592270067),
 .UNSPECIFIED.)
GEOMETRIC_REPRESENTATION_ITEM()
RATIONAL_B_SPLINE_SURFACE(((1.,0.705266242717945,1.00062243212993),(1.,
0.705584085909577,1.00062176089425),(1.,0.70618208945095,1.00062049800322),
(1.,0.706797508587931,1.00061919833315)))
REPRESENTATION_ITEM('')
SURFACE()
);
#2964=(
BOUNDED_SURFACE()
B_SPLINE_SURFACE(3,2,((#205862,#205863,#205864),(#205865,#205866,#205867),
(#205868,#205869,#205870),(#205871,#205872,#205873)),.UNSPECIFIED.,.F.,
 .F.,.F.)
B_SPLINE_SURFACE_WITH_KNOTS((4,4),(3,3),(0.,0.00039739442808661),(0.,1.),
 .UNSPECIFIED.)
GEOMETRIC_REPRESENTATION_ITEM()
RATIONAL_B_SPLINE_SURFACE(((1.,0.707106781186548,1.),(1.,0.706459846759103,
1.),(1.,0.705820510737282,1.),(1.,0.705498956110752,1.)))
REPRESENTATION_ITEM('')
SURFACE()
);
#2965=(
BOUNDED_SURFACE()
B_SPLINE_SURFACE(3,2,((#205879,#205880,#205881),(#205882,#205883,#205884),
(#205885,#205886,#205887),(#205888,#205889,#205890),(#205891,#205892,#205893),
(#205894,#205895,#205896)),.UNSPECIFIED.,.F.,.F.,.F.)
B_SPLINE_SURFACE_WITH_KNOTS((4,2,4),(3,3),(0.,0.000257953807872847,0.000515907615745694),
(0.,1.),.UNSPECIFIED.)
GEOMETRIC_REPRESENTATION_ITEM()
RATIONAL_B_SPLINE_SURFACE(((1.,0.87461970713939,1.),(1.,0.874834349678675,
1.),(1.,0.854686104158191,1.),(1.,0.79247659791475,1.),(1.,0.750887854595405,
1.),(1.,0.705585838031447,1.)))
REPRESENTATION_ITEM('')
SURFACE()
);
#2966=(
BOUNDED_SURFACE()
B_SPLINE_SURFACE(3,2,((#205902,#205903,#205904),(#205905,#205906,#205907),
(#205908,#205909,#205910),(#205911,#205912,#205913)),.UNSPECIFIED.,.F.,
 .F.,.F.)
B_SPLINE_SURFACE_WITH_KNOTS((4,4),(3,3),(-9.64939933512099E-18,0.000511815437699153),
(0.,1.00105881331513),.UNSPECIFIED.)
GEOMETRIC_REPRESENTATION_ITEM()
RATIONAL_B_SPLINE_SURFACE(((1.,0.706796661946555,1.00062089519675),(1.,
0.707430821225458,1.00061955228417),(1.,0.708058545830927,1.00061822299783),
(1.,0.70839450525293,1.00061751156121)))
REPRESENTATION_ITEM('')
SURFACE()
);
#2967=(
BOUNDED_SURFACE()
B_SPLINE_SURFACE(3,2,((#205915,#205916,#205917),(#205918,#205919,#205920),
(#205921,#205922,#205923),(#205924,#205925,#205926),(#205927,#205928,#205929),
(#205930,#205931,#205932)),.UNSPECIFIED.,.F.,.F.,.F.)
B_SPLINE_SURFACE_WITH_KNOTS((4,2,4),(3,3),(0.,0.00025691531753127,0.000513830635062539),
(0.,1.),.UNSPECIFIED.)
GEOMETRIC_REPRESENTATION_ITEM()
RATIONAL_B_SPLINE_SURFACE(((1.,0.705585838031426,1.),(1.,0.750902433542389,
1.),(1.,0.792329530083006,1.),(1.,0.854288401593708,1.),(1.,0.87499803112553,
1.),(1.,0.874619707139387,1.)))
REPRESENTATION_ITEM('')
SURFACE()
);
#2968=(
BOUNDED_SURFACE()
B_SPLINE_SURFACE(3,2,((#205938,#205939,#205940),(#205941,#205942,#205943),
(#205944,#205945,#205946),(#205947,#205948,#205949),(#205950,#205951,#205952),
(#205953,#205954,#205955)),.UNSPECIFIED.,.F.,.F.,.F.)
B_SPLINE_SURFACE_WITH_KNOTS((4,2,4),(3,3),(0.,0.000256592814262155,0.000513185628524311),
(0.,1.),.UNSPECIFIED.)
GEOMETRIC_REPRESENTATION_ITEM()
RATIONAL_B_SPLINE_SURFACE(((1.,0.708712527163685,1.),(1.,0.753780902614243,
1.),(1.,0.794538995768276,1.),(1.,0.855070770332059,1.),(1.,0.875018427444598,
1.),(1.,0.874619707139393,1.)))
REPRESENTATION_ITEM('')
SURFACE()
);
#2969=(
BOUNDED_SURFACE()
B_SPLINE_SURFACE(3,2,((#205957,#205958,#205959),(#205960,#205961,#205962),
(#205963,#205964,#205965),(#205966,#205967,#205968)),.UNSPECIFIED.,.F.,
 .F.,.F.)
B_SPLINE_SURFACE_WITH_KNOTS((4,4),(3,3),(0.,0.000511815072430395),(0.,1.00105598365835),
 .UNSPECIFIED.)
GEOMETRIC_REPRESENTATION_ITEM()
RATIONAL_B_SPLINE_SURFACE(((1.,0.70679749073384,1.00061923411674),(1.,0.706182062146739,
1.0006205338818),(1.,0.705584062769122,1.00062179683694),(1.,0.705266224770601,
1.00062246810041)))
REPRESENTATION_ITEM('')
SURFACE()
);
#2970=(
BOUNDED_SURFACE()
B_SPLINE_SURFACE(3,2,((#205974,#205975,#205976),(#205977,#205978,#205979),
(#205980,#205981,#205982),(#205983,#205984,#205985),(#205986,#205987,#205988),
(#205989,#205990,#205991)),.UNSPECIFIED.,.F.,.F.,.F.)
B_SPLINE_SURFACE_WITH_KNOTS((4,2,4),(3,3),(0.,0.000257652232350885,0.00051530446470177),
(0.,1.),.UNSPECIFIED.)
GEOMETRIC_REPRESENTATION_ITEM()
RATIONAL_B_SPLINE_SURFACE(((1.,0.874619707139382,1.),(1.,0.874861180430943,
1.),(1.,0.855455725920536,1.),(1.,0.794699358955577,1.),(1.,0.753768977788396,
1.),(1.,0.708712527163675,1.)))
REPRESENTATION_ITEM('')
SURFACE()
);
#2971=(
BOUNDED_SURFACE()
B_SPLINE_SURFACE(3,2,((#205997,#205998,#205999),(#206000,#206001,#206002),
(#206003,#206004,#206005),(#206006,#206007,#206008)),.UNSPECIFIED.,.F.,
 .F.,.F.)
B_SPLINE_SURFACE_WITH_KNOTS((4,4),(3,3),(0.,0.000397394373651913),(0.,1.),
 .UNSPECIFIED.)
GEOMETRIC_REPRESENTATION_ITEM()
RATIONAL_B_SPLINE_SURFACE(((1.,0.707106781186548,1.),(1.,0.707752587915884,
1.),(1.,0.708377654540707,1.),(1.,0.708689770883326,1.)))
REPRESENTATION_ITEM('')
SURFACE()
);
#2972=(
BOUNDED_SURFACE()
B_SPLINE_SURFACE(3,2,((#206010,#206011,#206012),(#206013,#206014,#206015),
(#206016,#206017,#206018),(#206019,#206020,#206021)),.UNSPECIFIED.,.F.,
 .F.,.F.)
B_SPLINE_SURFACE_WITH_KNOTS((4,4),(3,3),(0.,0.000511815456479787),(0.,1.00105873159594),
 .UNSPECIFIED.)
GEOMETRIC_REPRESENTATION_ITEM()
RATIONAL_B_SPLINE_SURFACE(((1.,0.708394529057491,1.00061746385127),(1.,
0.708058564168059,1.00061817524456),(1.,0.707430835373237,1.00061950443718),
(1.,0.706796685881553,1.00062084722538)))
REPRESENTATION_ITEM('')
SURFACE()
);
#2973=(
BOUNDED_SURFACE()
B_SPLINE_SURFACE(3,2,((#206027,#206028,#206029),(#206030,#206031,#206032),
(#206033,#206034,#206035),(#206036,#206037,#206038)),.UNSPECIFIED.,.F.,
 .F.,.F.)
B_SPLINE_SURFACE_WITH_KNOTS((4,4),(3,3),(0.,0.000397394465448302),(0.,1.),
 .UNSPECIFIED.)
GEOMETRIC_REPRESENTATION_ITEM()
RATIONAL_B_SPLINE_SURFACE(((1.,0.705498956110742,1.),(1.,0.705821764811801,
1.),(1.,0.706461952521133,1.),(1.,0.707106781186548,1.)))
REPRESENTATION_ITEM('')
SURFACE()
);
#2974=(
BOUNDED_SURFACE()
B_SPLINE_SURFACE(3,2,((#206044,#206045,#206046),(#206047,#206048,#206049),
(#206050,#206051,#206052),(#206053,#206054,#206055)),.UNSPECIFIED.,.F.,
 .F.,.F.)
B_SPLINE_SURFACE_WITH_KNOTS((4,4),(3,3),(0.,0.000397394410828734),(0.,1.),
 .UNSPECIFIED.)
GEOMETRIC_REPRESENTATION_ITEM()
RATIONAL_B_SPLINE_SURFACE(((1.,0.708689770883308,1.),(1.,0.708376440034539,
1.),(1.,0.70775049869839,1.),(1.,0.707106781186548,1.)))
REPRESENTATION_ITEM('')
SURFACE()
);
#2975=(
BOUNDED_SURFACE()
B_SPLINE_SURFACE(3,2,((#206061,#206062,#206063),(#206064,#206065,#206066),
(#206067,#206068,#206069),(#206070,#206071,#206072)),.UNSPECIFIED.,.F.,
 .F.,.F.)
B_SPLINE_SURFACE_WITH_KNOTS((4,4),(3,3),(0.,0.000511815090126186),(0.,1.00105592270023),
 .UNSPECIFIED.)
GEOMETRIC_REPRESENTATION_ITEM()
RATIONAL_B_SPLINE_SURFACE(((1.,0.705266242718059,1.00062243212967),(1.,
0.705584085909722,1.00062176089399),(1.,0.706182089451054,1.00062049800296),
(1.,0.706797508588071,1.00061919833289)))
REPRESENTATION_ITEM('')
SURFACE()
);
#2976=(
BOUNDED_SURFACE()
B_SPLINE_SURFACE(3,2,((#206074,#206075,#206076),(#206077,#206078,#206079),
(#206080,#206081,#206082),(#206083,#206084,#206085)),.UNSPECIFIED.,.F.,
 .F.,.F.)
B_SPLINE_SURFACE_WITH_KNOTS((4,4),(3,3),(-5.52943107967607E-18,0.000397394428086622),
(0.,1.),.UNSPECIFIED.)
GEOMETRIC_REPRESENTATION_ITEM()
RATIONAL_B_SPLINE_SURFACE(((1.,0.707106781186548,1.),(1.,0.706459846759108,
1.),(1.,0.70582051073728,1.),(1.,0.705498956110745,1.)))
REPRESENTATION_ITEM('')
SURFACE()
);
#2977=(
BOUNDED_SURFACE()
B_SPLINE_SURFACE(3,2,((#206091,#206092,#206093),(#206094,#206095,#206096),
(#206097,#206098,#206099),(#206100,#206101,#206102),(#206103,#206104,#206105),
(#206106,#206107,#206108)),.UNSPECIFIED.,.F.,.F.,.F.)
B_SPLINE_SURFACE_WITH_KNOTS((4,2,4),(3,3),(0.,0.000257953807872851,0.000515907615745702),
(0.,1.),.UNSPECIFIED.)
GEOMETRIC_REPRESENTATION_ITEM()
RATIONAL_B_SPLINE_SURFACE(((1.,0.874619707139392,1.),(1.,0.874834349679009,
1.),(1.,0.854686104157774,1.),(1.,0.792476597915158,1.),(1.,0.750887854595105,
1.),(1.,0.705585838031436,1.)))
REPRESENTATION_ITEM('')
SURFACE()
);
#2978=(
BOUNDED_SURFACE()
B_SPLINE_SURFACE(3,2,((#206114,#206115,#206116),(#206117,#206118,#206119),
(#206120,#206121,#206122),(#206123,#206124,#206125)),.UNSPECIFIED.,.F.,
 .F.,.F.)
B_SPLINE_SURFACE_WITH_KNOTS((4,4),(3,3),(0.,0.000511815437699149),(0.,1.0010588133169),
 .UNSPECIFIED.)
GEOMETRIC_REPRESENTATION_ITEM()
RATIONAL_B_SPLINE_SURFACE(((1.,0.706796661946038,1.00062089519778),(1.,
0.707430821224916,1.0006195522852),(1.,0.708058545830393,1.00061822299886),
(1.,0.708394505252432,1.00061751156224)))
REPRESENTATION_ITEM('')
SURFACE()
);
#2979=(
BOUNDED_SURFACE()
B_SPLINE_SURFACE(3,2,((#206127,#206128,#206129),(#206130,#206131,#206132),
(#206133,#206134,#206135),(#206136,#206137,#206138),(#206139,#206140,#206141),
(#206142,#206143,#206144)),.UNSPECIFIED.,.F.,.F.,.F.)
B_SPLINE_SURFACE_WITH_KNOTS((4,2,4),(3,3),(0.,0.000256915317531261,0.000513830635062523),
(0.,1.),.UNSPECIFIED.)
GEOMETRIC_REPRESENTATION_ITEM()
RATIONAL_B_SPLINE_SURFACE(((1.,0.705585838031425,1.),(1.,0.750902433543488,
1.),(1.,0.792329530081549,1.),(1.,0.854288401595205,1.),(1.,0.874998031124371,
1.),(1.,0.874619707139389,1.)))
REPRESENTATION_ITEM('')
SURFACE()
);
#2980=(
BOUNDED_SURFACE()
B_SPLINE_SURFACE(3,2,((#206150,#206151,#206152),(#206153,#206154,#206155),
(#206156,#206157,#206158),(#206159,#206160,#206161),(#206162,#206163,#206164),
(#206165,#206166,#206167)),.UNSPECIFIED.,.F.,.F.,.F.)
B_SPLINE_SURFACE_WITH_KNOTS((4,2,4),(3,3),(0.,0.000256592814262158,0.000513185628524316),
(0.,1.),.UNSPECIFIED.)
GEOMETRIC_REPRESENTATION_ITEM()
RATIONAL_B_SPLINE_SURFACE(((1.,0.708712527163672,1.),(1.,0.753780902613422,
1.),(1.,0.794538995769399,1.),(1.,0.855070770330892,1.),(1.,0.875018427445483,
1.),(1.,0.874619707139387,1.)))
REPRESENTATION_ITEM('')
SURFACE()
);
#2981=(
BOUNDED_SURFACE()
B_SPLINE_SURFACE(3,2,((#206169,#206170,#206171),(#206172,#206173,#206174),
(#206175,#206176,#206177),(#206178,#206179,#206180)),.UNSPECIFIED.,.F.,
 .F.,.F.)
B_SPLINE_SURFACE_WITH_KNOTS((4,4),(3,3),(0.,0.000511815072430397),(0.,1.00105598366041),
 .UNSPECIFIED.)
GEOMETRIC_REPRESENTATION_ITEM()
RATIONAL_B_SPLINE_SURFACE(((1.,0.706797490733247,1.00061923411795),(1.,
0.706182062146158,1.00062053388302),(1.,0.705584062768489,1.00062179683816),
(1.,0.705266224770021,1.00062246810163)))
REPRESENTATION_ITEM('')
SURFACE()
);
#2982=(
BOUNDED_SURFACE()
B_SPLINE_SURFACE(3,2,((#206186,#206187,#206188),(#206189,#206190,#206191),
(#206192,#206193,#206194),(#206195,#206196,#206197),(#206198,#206199,#206200),
(#206201,#206202,#206203)),.UNSPECIFIED.,.F.,.F.,.F.)
B_SPLINE_SURFACE_WITH_KNOTS((4,2,4),(3,3),(0.,0.000257652232350886,0.000515304464701773),
(0.,1.),.UNSPECIFIED.)
GEOMETRIC_REPRESENTATION_ITEM()
RATIONAL_B_SPLINE_SURFACE(((1.,0.874619707139387,1.),(1.,0.874861180430777,
1.),(1.,0.85545572592079,1.),(1.,0.794699358955371,1.),(1.,0.753768977788547,
1.),(1.,0.708712527163673,1.)))
REPRESENTATION_ITEM('')
SURFACE()
);
#2983=(
BOUNDED_SURFACE()
B_SPLINE_SURFACE(3,2,((#206209,#206210,#206211),(#206212,#206213,#206214),
(#206215,#206216,#206217),(#206218,#206219,#206220)),.UNSPECIFIED.,.F.,
 .F.,.F.)
B_SPLINE_SURFACE_WITH_KNOTS((4,4),(3,3),(0.,0.000397394373651913),(0.,1.),
 .UNSPECIFIED.)
GEOMETRIC_REPRESENTATION_ITEM()
RATIONAL_B_SPLINE_SURFACE(((1.,0.707106781186536,1.),(1.,0.707752587915919,
1.),(1.,0.70837765454067,1.),(1.,0.708689770883331,1.)))
REPRESENTATION_ITEM('')
SURFACE()
);
#2984=(
BOUNDED_SURFACE()
B_SPLINE_SURFACE(3,2,((#206222,#206223,#206224),(#206225,#206226,#206227),
(#206228,#206229,#206230),(#206231,#206232,#206233)),.UNSPECIFIED.,.F.,
 .F.,.F.)
B_SPLINE_SURFACE_WITH_KNOTS((4,4),(3,3),(0.,0.000511815456479785),(0.,1.00105873159934),
 .UNSPECIFIED.)
GEOMETRIC_REPRESENTATION_ITEM()
RATIONAL_B_SPLINE_SURFACE(((1.,0.708394529056502,1.00061746385326),(1.,
0.708058564167077,1.00061817524654),(1.,0.70743083537222,1.00061950443917),
(1.,0.706796685880547,1.00062084722738)))
REPRESENTATION_ITEM('')
SURFACE()
);
#2985=(
BOUNDED_SURFACE()
B_SPLINE_SURFACE(3,2,((#206239,#206240,#206241),(#206242,#206243,#206244),
(#206245,#206246,#206247),(#206248,#206249,#206250)),.UNSPECIFIED.,.F.,
 .F.,.F.)
B_SPLINE_SURFACE_WITH_KNOTS((4,4),(3,3),(0.,0.000397394465448304),(0.,1.),
 .UNSPECIFIED.)
GEOMETRIC_REPRESENTATION_ITEM()
RATIONAL_B_SPLINE_SURFACE(((1.,0.705498956110752,1.),(1.,0.705821764811803,
1.),(1.,0.706461952521127,1.),(1.,0.707106781186548,1.)))
REPRESENTATION_ITEM('')
SURFACE()
);
#2986=(
BOUNDED_SURFACE()
B_SPLINE_SURFACE(3,2,((#206256,#206257,#206258),(#206259,#206260,#206261),
(#206262,#206263,#206264),(#206265,#206266,#206267)),.UNSPECIFIED.,.F.,
 .F.,.F.)
B_SPLINE_SURFACE_WITH_KNOTS((4,4),(3,3),(0.,0.000397394410828736),(0.,1.),
 .UNSPECIFIED.)
GEOMETRIC_REPRESENTATION_ITEM()
RATIONAL_B_SPLINE_SURFACE(((1.,0.70868977088333,1.),(1.,0.708376440034522,
1.),(1.,0.707750498698396,1.),(1.,0.707106781186548,1.)))
REPRESENTATION_ITEM('')
SURFACE()
);
#2987=(
BOUNDED_SURFACE()
B_SPLINE_SURFACE(3,2,((#206273,#206274,#206275),(#206276,#206277,#206278),
(#206279,#206280,#206281),(#206282,#206283,#206284)),.UNSPECIFIED.,.F.,
 .F.,.F.)
B_SPLINE_SURFACE_WITH_KNOTS((4,4),(3,3),(0.,0.000511815090126171),(0.,1.00105592270543),
 .UNSPECIFIED.)
GEOMETRIC_REPRESENTATION_ITEM()
RATIONAL_B_SPLINE_SURFACE(((1.,0.705266242716512,1.00062243213275),(1.,
0.705584085908209,1.00062176089706),(1.,0.706182089449527,1.00062049800603),
(1.,0.706797508586535,1.00061919833595)))
REPRESENTATION_ITEM('')
SURFACE()
);
#2988=(
BOUNDED_SURFACE()
B_SPLINE_SURFACE(3,2,((#206286,#206287,#206288),(#206289,#206290,#206291),
(#206292,#206293,#206294),(#206295,#206296,#206297)),.UNSPECIFIED.,.F.,
 .F.,.F.)
B_SPLINE_SURFACE_WITH_KNOTS((4,4),(3,3),(0.,0.000397394428086614),(0.,1.),
 .UNSPECIFIED.)
GEOMETRIC_REPRESENTATION_ITEM()
RATIONAL_B_SPLINE_SURFACE(((1.,0.707106781186548,1.),(1.,0.706459846759078,
1.),(1.,0.705820510737289,1.),(1.,0.705498956110736,1.)))
REPRESENTATION_ITEM('')
SURFACE()
);
#2989=(
BOUNDED_SURFACE()
B_SPLINE_SURFACE(3,2,((#206303,#206304,#206305),(#206306,#206307,#206308),
(#206309,#206310,#206311),(#206312,#206313,#206314),(#206315,#206316,#206317),
(#206318,#206319,#206320)),.UNSPECIFIED.,.F.,.F.,.F.)
B_SPLINE_SURFACE_WITH_KNOTS((4,2,4),(3,3),(0.,0.000257953807872845,0.00051590761574569),
(0.,1.),.UNSPECIFIED.)
GEOMETRIC_REPRESENTATION_ITEM()
RATIONAL_B_SPLINE_SURFACE(((1.,0.874619707139387,1.),(1.,0.87483434967959,
1.),(1.,0.854686104157006,1.),(1.,0.792476597915929,1.),(1.,0.750887854594532,
1.),(1.,0.705585838031438,1.)))
REPRESENTATION_ITEM('')
SURFACE()
);
#2990=(
BOUNDED_SURFACE()
B_SPLINE_SURFACE(3,2,((#206326,#206327,#206328),(#206329,#206330,#206331),
(#206332,#206333,#206334),(#206335,#206336,#206337)),.UNSPECIFIED.,.F.,
 .F.,.F.)
B_SPLINE_SURFACE_WITH_KNOTS((4,4),(3,3),(0.,0.000511815437699149),(0.,1.0010588133194),
 .UNSPECIFIED.)
GEOMETRIC_REPRESENTATION_ITEM()
RATIONAL_B_SPLINE_SURFACE(((1.,0.706796661945307,1.00062089519925),(1.,
0.707430821224188,1.00061955228667),(1.,0.708058545829719,1.00061822300032),
(1.,0.708394505251694,1.0006175115637)))
REPRESENTATION_ITEM('')
SURFACE()
);
#2991=(
BOUNDED_SURFACE()
B_SPLINE_SURFACE(3,2,((#206339,#206340,#206341),(#206342,#206343,#206344),
(#206345,#206346,#206347),(#206348,#206349,#206350),(#206351,#206352,#206353),
(#206354,#206355,#206356)),.UNSPECIFIED.,.F.,.F.,.F.)
B_SPLINE_SURFACE_WITH_KNOTS((4,2,4),(3,3),(0.,0.000256915317531267,0.000513830635062534),
(0.,1.),.UNSPECIFIED.)
GEOMETRIC_REPRESENTATION_ITEM()
RATIONAL_B_SPLINE_SURFACE(((1.,0.705585838031461,1.),(1.,0.750902433542758,
1.),(1.,0.792329530082508,1.),(1.,0.854288401594206,1.),(1.,0.874998031125127,
1.),(1.,0.8746197071394,1.)))
REPRESENTATION_ITEM('')
SURFACE()
);
#2992=(
BOUNDED_SURFACE()
B_SPLINE_SURFACE(3,2,((#206362,#206363,#206364),(#206365,#206366,#206367),
(#206368,#206369,#206370),(#206371,#206372,#206373),(#206374,#206375,#206376),
(#206377,#206378,#206379)),.UNSPECIFIED.,.F.,.F.,.F.)
B_SPLINE_SURFACE_WITH_KNOTS((4,2,4),(3,3),(0.,0.000256592814262156,0.000513185628524312),
(0.,1.),.UNSPECIFIED.)
GEOMETRIC_REPRESENTATION_ITEM()
RATIONAL_B_SPLINE_SURFACE(((1.,0.708712527163667,1.),(1.,0.753780902613713,
1.),(1.,0.794538995769065,1.),(1.,0.855070770331245,1.),(1.,0.875018427445222,
1.),(1.,0.874619707139387,1.)))
REPRESENTATION_ITEM('')
SURFACE()
);
#2993=(
BOUNDED_SURFACE()
B_SPLINE_SURFACE(3,2,((#206381,#206382,#206383),(#206384,#206385,#206386),
(#206387,#206388,#206389),(#206390,#206391,#206392)),.UNSPECIFIED.,.F.,
 .F.,.F.)
B_SPLINE_SURFACE_WITH_KNOTS((4,4),(3,3),(0.,0.000511815072430405),(0.,1.00105598366104),
 .UNSPECIFIED.)
GEOMETRIC_REPRESENTATION_ITEM()
RATIONAL_B_SPLINE_SURFACE(((1.,0.70679749073305,1.00061923411833),(1.,0.706182062145971,
1.00062053388339),(1.,0.705584062768321,1.00062179683854),(1.,0.705266224769805,
1.000622468102)))
REPRESENTATION_ITEM('')
SURFACE()
);
#2994=(
BOUNDED_SURFACE()
B_SPLINE_SURFACE(3,2,((#206398,#206399,#206400),(#206401,#206402,#206403),
(#206404,#206405,#206406),(#206407,#206408,#206409),(#206410,#206411,#206412),
(#206413,#206414,#206415)),.UNSPECIFIED.,.F.,.F.,.F.)
B_SPLINE_SURFACE_WITH_KNOTS((4,2,4),(3,3),(-2.80537312130624E-18,0.000257652232350884,
0.000515304464701771),(0.,1.),.UNSPECIFIED.)
GEOMETRIC_REPRESENTATION_ITEM()
RATIONAL_B_SPLINE_SURFACE(((1.,0.874619707139388,1.),(1.,0.874861180430588,
1.),(1.,0.855455725920997,1.),(1.,0.794699358955135,1.),(1.,0.753768977788717,
1.),(1.,0.708712527163664,1.)))
REPRESENTATION_ITEM('')
SURFACE()
);
#2995=(
BOUNDED_SURFACE()
B_SPLINE_SURFACE(3,2,((#206421,#206422,#206423),(#206424,#206425,#206426),
(#206427,#206428,#206429),(#206430,#206431,#206432)),.UNSPECIFIED.,.F.,
 .F.,.F.)
B_SPLINE_SURFACE_WITH_KNOTS((4,4),(3,3),(-7.64362531602281E-18,0.000397394373651905),
(0.,1.),.UNSPECIFIED.)
GEOMETRIC_REPRESENTATION_ITEM()
RATIONAL_B_SPLINE_SURFACE(((1.,0.707106781186548,1.),(1.,0.707752587915893,
1.),(1.,0.708377654540694,1.),(1.,0.708689770883325,1.)))
REPRESENTATION_ITEM('')
SURFACE()
);
#2996=(
BOUNDED_SURFACE()
B_SPLINE_SURFACE(3,2,((#206434,#206435,#206436),(#206437,#206438,#206439),
(#206440,#206441,#206442),(#206443,#206444,#206445)),.UNSPECIFIED.,.F.,
 .F.,.F.)
B_SPLINE_SURFACE_WITH_KNOTS((4,4),(3,3),(0.,0.000511815456479789),(0.,1.0010587316006),
 .UNSPECIFIED.)
GEOMETRIC_REPRESENTATION_ITEM()
RATIONAL_B_SPLINE_SURFACE(((1.,0.708394529056127,1.00061746385399),(1.,
0.708058564166706,1.00061817524728),(1.,0.707430835371847,1.00061950443991),
(1.,0.706796685880188,1.00062084722812)))
REPRESENTATION_ITEM('')
SURFACE()
);
#2997=(
BOUNDED_SURFACE()
B_SPLINE_SURFACE(3,2,((#206451,#206452,#206453),(#206454,#206455,#206456),
(#206457,#206458,#206459),(#206460,#206461,#206462)),.UNSPECIFIED.,.F.,
 .F.,.F.)
B_SPLINE_SURFACE_WITH_KNOTS((4,4),(3,3),(-6.50521303491303E-18,0.000397394465448314),
(0.,1.),.UNSPECIFIED.)
GEOMETRIC_REPRESENTATION_ITEM()
RATIONAL_B_SPLINE_SURFACE(((1.,0.705498956110783,1.),(1.,0.70582176481173,
1.),(1.,0.706461952521176,1.),(1.,0.707106781186546,1.)))
REPRESENTATION_ITEM('')
SURFACE()
);
#2998=(
BOUNDED_SURFACE()
B_SPLINE_SURFACE(3,2,((#206468,#206469,#206470),(#206471,#206472,#206473),
(#206474,#206475,#206476),(#206477,#206478,#206479)),.UNSPECIFIED.,.F.,
 .F.,.F.)
B_SPLINE_SURFACE_WITH_KNOTS((4,4),(3,3),(0.,0.000397394410828748),(0.,1.),
 .UNSPECIFIED.)
GEOMETRIC_REPRESENTATION_ITEM()
RATIONAL_B_SPLINE_SURFACE(((1.,0.708689770883336,1.),(1.,0.708376440034494,
1.),(1.,0.707750498698415,1.),(1.,0.707106781186548,1.)))
REPRESENTATION_ITEM('')
SURFACE()
);
#2999=(
BOUNDED_SURFACE()
B_SPLINE_SURFACE(3,2,((#206485,#206486,#206487),(#206488,#206489,#206490),
(#206491,#206492,#206493),(#206494,#206495,#206496)),.UNSPECIFIED.,.F.,
 .F.,.F.)
B_SPLINE_SURFACE_WITH_KNOTS((4,4),(3,3),(-6.42389787197661E-18,0.000511815090126191),
(0.,1.00105592270157),.UNSPECIFIED.)
GEOMETRIC_REPRESENTATION_ITEM()
RATIONAL_B_SPLINE_SURFACE(((1.,0.705266242717654,1.00062243213047),(1.,
0.705584085909314,1.00062176089479),(1.,0.706182089450723,1.00062049800376),
(1.,0.706797508587648,1.00061919833368)))
REPRESENTATION_ITEM('')
SURFACE()
);
#3000=(
BOUNDED_SURFACE()
B_SPLINE_SURFACE(3,2,((#206498,#206499,#206500),(#206501,#206502,#206503),
(#206504,#206505,#206506),(#206507,#206508,#206509)),.UNSPECIFIED.,.F.,
 .F.,.F.)
B_SPLINE_SURFACE_WITH_KNOTS((4,4),(3,3),(0.,0.000397394428086633),(0.,1.),
 .UNSPECIFIED.)
GEOMETRIC_REPRESENTATION_ITEM()
RATIONAL_B_SPLINE_SURFACE(((1.,0.707106781186556,1.),(1.,0.706459846759107,
1.),(1.,0.705820510737253,1.),(1.,0.705498956110758,1.)))
REPRESENTATION_ITEM('')
SURFACE()
);
#3001=(
BOUNDED_SURFACE()
B_SPLINE_SURFACE(3,2,((#206515,#206516,#206517),(#206518,#206519,#206520),
(#206521,#206522,#206523),(#206524,#206525,#206526),(#206527,#206528,#206529),
(#206530,#206531,#206532)),.UNSPECIFIED.,.F.,.F.,.F.)
B_SPLINE_SURFACE_WITH_KNOTS((4,2,4),(3,3),(0.,0.000257953807872838,0.000515907615745676),
(0.,1.),.UNSPECIFIED.)
GEOMETRIC_REPRESENTATION_ITEM()
RATIONAL_B_SPLINE_SURFACE(((1.,0.874619707139395,1.),(1.,0.874834349679273,
1.),(1.,0.854686104157422,1.),(1.,0.792476597915473,1.),(1.,0.750887854594883,
1.),(1.,0.705585838031443,1.)))
REPRESENTATION_ITEM('')
SURFACE()
);
#3002=(
BOUNDED_SURFACE()
B_SPLINE_SURFACE(3,2,((#206538,#206539,#206540),(#206541,#206542,#206543),
(#206544,#206545,#206546),(#206547,#206548,#206549)),.UNSPECIFIED.,.F.,
 .F.,.F.)
B_SPLINE_SURFACE_WITH_KNOTS((4,4),(3,3),(0.,0.000511815437699146),(0.,1.00105881331723),
 .UNSPECIFIED.)
GEOMETRIC_REPRESENTATION_ITEM()
RATIONAL_B_SPLINE_SURFACE(((1.,0.70679666194594,1.00062089519798),(1.,0.707430821224803,
1.0006195522854),(1.,0.70805854583036,1.00061822299905),(1.,0.70839450525233,
1.00061751156243)))
REPRESENTATION_ITEM('')
SURFACE()
);
#3003=(
BOUNDED_SURFACE()
B_SPLINE_SURFACE(3,2,((#206551,#206552,#206553),(#206554,#206555,#206556),
(#206557,#206558,#206559),(#206560,#206561,#206562),(#206563,#206564,#206565),
(#206566,#206567,#206568)),.UNSPECIFIED.,.F.,.F.,.F.)
B_SPLINE_SURFACE_WITH_KNOTS((4,2,4),(3,3),(0.,0.000256915317531265,0.00051383063506253),
(0.,1.),.UNSPECIFIED.)
GEOMETRIC_REPRESENTATION_ITEM()
RATIONAL_B_SPLINE_SURFACE(((1.,0.705585838031446,1.),(1.,0.750902433543011,
1.),(1.,0.792329530082201,1.),(1.,0.854288401594521,1.),(1.,0.874998031124925,
1.),(1.,0.874619707139403,1.)))
REPRESENTATION_ITEM('')
SURFACE()
);
#3004=(
BOUNDED_SURFACE()
B_SPLINE_SURFACE(3,2,((#206574,#206575,#206576),(#206577,#206578,#206579),
(#206580,#206581,#206582),(#206583,#206584,#206585),(#206586,#206587,#206588),
(#206589,#206590,#206591)),.UNSPECIFIED.,.F.,.F.,.F.)
B_SPLINE_SURFACE_WITH_KNOTS((4,2,4),(3,3),(0.,0.000256592814262155,0.00051318562852431),
(0.,1.),.UNSPECIFIED.)
GEOMETRIC_REPRESENTATION_ITEM()
RATIONAL_B_SPLINE_SURFACE(((1.,0.708712527163695,1.),(1.,0.753780902613568,
1.),(1.,0.794538995769177,1.),(1.,0.855070770331137,1.),(1.,0.875018427445306,
1.),(1.,0.874619707139389,1.)))
REPRESENTATION_ITEM('')
SURFACE()
);
#3005=(
BOUNDED_SURFACE()
B_SPLINE_SURFACE(3,2,((#206593,#206594,#206595),(#206596,#206597,#206598),
(#206599,#206600,#206601),(#206602,#206603,#206604)),.UNSPECIFIED.,.F.,
 .F.,.F.)
B_SPLINE_SURFACE_WITH_KNOTS((4,4),(3,3),(-2.71050543121376E-20,0.00051181507243041),
(0.,1.00105598366241),.UNSPECIFIED.)
GEOMETRIC_REPRESENTATION_ITEM()
RATIONAL_B_SPLINE_SURFACE(((1.,0.706797490732659,1.00061923411913),(1.,
0.706182062145589,1.00062053388419),(1.,0.705584062767944,1.00062179683934),
(1.,0.70526622476939,1.00062246810281)))
REPRESENTATION_ITEM('')
SURFACE()
);
#3006=(
BOUNDED_SURFACE()
B_SPLINE_SURFACE(3,2,((#206610,#206611,#206612),(#206613,#206614,#206615),
(#206616,#206617,#206618),(#206619,#206620,#206621),(#206622,#206623,#206624),
(#206625,#206626,#206627)),.UNSPECIFIED.,.F.,.F.,.F.)
B_SPLINE_SURFACE_WITH_KNOTS((4,2,4),(3,3),(-9.32413868337534E-18,0.000257652232350879,
0.000515304464701767),(0.,1.),.UNSPECIFIED.)
GEOMETRIC_REPRESENTATION_ITEM()
RATIONAL_B_SPLINE_SURFACE(((1.,0.87461970713939,1.),(1.,0.874861180430825,
1.),(1.,0.855455725920677,1.),(1.,0.794699358955439,1.),(1.,0.753768977788503,
1.),(1.,0.708712527163652,1.)))
REPRESENTATION_ITEM('')
SURFACE()
);
#3007=(
BOUNDED_SURFACE()
B_SPLINE_SURFACE(3,2,((#206633,#206634,#206635),(#206636,#206637,#206638),
(#206639,#206640,#206641),(#206642,#206643,#206644)),.UNSPECIFIED.,.F.,
 .F.,.F.)
B_SPLINE_SURFACE_WITH_KNOTS((4,4),(3,3),(0.,0.000397394373651905),(0.,1.),
 .UNSPECIFIED.)
GEOMETRIC_REPRESENTATION_ITEM()
RATIONAL_B_SPLINE_SURFACE(((1.,0.707106781186555,1.),(1.,0.707752587915883,
1.),(1.,0.708377654540676,1.),(1.,0.708689770883327,1.)))
REPRESENTATION_ITEM('')
SURFACE()
);
#3008=(
BOUNDED_SURFACE()
B_SPLINE_SURFACE(3,2,((#206646,#206647,#206648),(#206649,#206650,#206651),
(#206652,#206653,#206654),(#206655,#206656,#206657)),.UNSPECIFIED.,.F.,
 .F.,.F.)
B_SPLINE_SURFACE_WITH_KNOTS((4,4),(3,3),(0.,0.000511815456479779),(0.,1.00105873160079),
 .UNSPECIFIED.)
GEOMETRIC_REPRESENTATION_ITEM()
RATIONAL_B_SPLINE_SURFACE(((1.,0.708394529056081,1.0006174638541),(1.,0.708058564166629,
1.00061817524739),(1.,0.70743083537183,1.00061950444001),(1.,0.706796685880126,
1.00062084722823)))
REPRESENTATION_ITEM('')
SURFACE()
);
#3009=(
BOUNDED_SURFACE()
B_SPLINE_SURFACE(3,2,((#206663,#206664,#206665),(#206666,#206667,#206668),
(#206669,#206670,#206671),(#206672,#206673,#206674)),.UNSPECIFIED.,.F.,
 .F.,.F.)
B_SPLINE_SURFACE_WITH_KNOTS((4,4),(3,3),(0.,0.000397394465448301),(0.,1.),
 .UNSPECIFIED.)
GEOMETRIC_REPRESENTATION_ITEM()
RATIONAL_B_SPLINE_SURFACE(((1.,0.705498956110756,1.),(1.,0.70582176481178,
1.),(1.,0.706461952521141,1.),(1.,0.707106781186548,1.)))
REPRESENTATION_ITEM('')
SURFACE()
);
#3010=(
BOUNDED_SURFACE()
B_SPLINE_SURFACE(3,2,((#206680,#206681,#206682),(#206683,#206684,#206685),
(#206686,#206687,#206688),(#206689,#206690,#206691)),.UNSPECIFIED.,.F.,
 .F.,.F.)
B_SPLINE_SURFACE_WITH_KNOTS((4,4),(3,3),(0.,0.000397394410828731),(0.,1.),
 .UNSPECIFIED.)
GEOMETRIC_REPRESENTATION_ITEM()
RATIONAL_B_SPLINE_SURFACE(((1.,0.708689770883319,1.),(1.,0.708376440034476,
1.),(1.,0.707750498698424,1.),(1.,0.707106781186548,1.)))
REPRESENTATION_ITEM('')
SURFACE()
);
#3011=(
BOUNDED_SURFACE()
B_SPLINE_SURFACE(3,2,((#206697,#206698,#206699),(#206700,#206701,#206702),
(#206703,#206704,#206705),(#206706,#206707,#206708)),.UNSPECIFIED.,.F.,
 .F.,.F.)
B_SPLINE_SURFACE_WITH_KNOTS((4,4),(3,3),(0.,0.000511815090126184),(0.,1.00105592270507),
 .UNSPECIFIED.)
GEOMETRIC_REPRESENTATION_ITEM()
RATIONAL_B_SPLINE_SURFACE(((1.,0.705266242716637,1.00062243213253),(1.,
0.705584085908299,1.00062176089685),(1.,0.706182089449661,1.00062049800581),
(1.,0.70679750858664,1.00061919833573)))
REPRESENTATION_ITEM('')
SURFACE()
);
#3012=(
BOUNDED_SURFACE()
B_SPLINE_SURFACE(3,2,((#206710,#206711,#206712),(#206713,#206714,#206715),
(#206716,#206717,#206718),(#206719,#206720,#206721)),.UNSPECIFIED.,.F.,
 .F.,.F.)
B_SPLINE_SURFACE_WITH_KNOTS((4,4),(3,3),(0.,0.000397394428086631),(0.,1.),
 .UNSPECIFIED.)
GEOMETRIC_REPRESENTATION_ITEM()
RATIONAL_B_SPLINE_SURFACE(((1.,0.707106781186548,1.),(1.,0.706459846759093,
1.),(1.,0.705820510737288,1.),(1.,0.705498956110764,1.)))
REPRESENTATION_ITEM('')
SURFACE()
);
#3013=(
BOUNDED_SURFACE()
B_SPLINE_SURFACE(3,2,((#206727,#206728,#206729),(#206730,#206731,#206732),
(#206733,#206734,#206735),(#206736,#206737,#206738),(#206739,#206740,#206741),
(#206742,#206743,#206744)),.UNSPECIFIED.,.F.,.F.,.F.)
B_SPLINE_SURFACE_WITH_KNOTS((4,2,4),(3,3),(0.,0.000257953807872847,0.000515907615745693),
(0.,1.),.UNSPECIFIED.)
GEOMETRIC_REPRESENTATION_ITEM()
RATIONAL_B_SPLINE_SURFACE(((1.,0.874619707139398,1.),(1.,0.874834349679205,
1.),(1.,0.854686104157519,1.),(1.,0.792476597915395,1.),(1.,0.750887854594947,
1.),(1.,0.705585838031442,1.)))
REPRESENTATION_ITEM('')
SURFACE()
);
#3014=(
BOUNDED_SURFACE()
B_SPLINE_SURFACE(3,2,((#206750,#206751,#206752),(#206753,#206754,#206755),
(#206756,#206757,#206758),(#206759,#206760,#206761)),.UNSPECIFIED.,.F.,
 .F.,.F.)
B_SPLINE_SURFACE_WITH_KNOTS((4,4),(3,3),(0.,0.000511815437699154),(0.,1.00105881331611),
 .UNSPECIFIED.)
GEOMETRIC_REPRESENTATION_ITEM()
RATIONAL_B_SPLINE_SURFACE(((1.,0.706796661946269,1.00062089519732),(1.,
0.707430821225167,1.00061955228474),(1.,0.708058545830613,1.0006182229984),
(1.,0.708394505252643,1.00061751156178)))
REPRESENTATION_ITEM('')
SURFACE()
);
#3015=(
BOUNDED_SURFACE()
B_SPLINE_SURFACE(3,2,((#206763,#206764,#206765),(#206766,#206767,#206768),
(#206769,#206770,#206771),(#206772,#206773,#206774),(#206775,#206776,#206777),
(#206778,#206779,#206780)),.UNSPECIFIED.,.F.,.F.,.F.)
B_SPLINE_SURFACE_WITH_KNOTS((4,2,4),(3,3),(9.97465998686664E-18,0.000256915317531272,
0.000513830635062533),(0.,1.),.UNSPECIFIED.)
GEOMETRIC_REPRESENTATION_ITEM()
RATIONAL_B_SPLINE_SURFACE(((1.,0.705585838031435,1.),(1.,0.750902433542796,
1.),(1.,0.792329530082492,1.),(1.,0.854288401594256,1.),(1.,0.874998031125097,
1.),(1.,0.874619707139405,1.)))
REPRESENTATION_ITEM('')
SURFACE()
);
#3016=(
BOUNDED_SURFACE()
B_SPLINE_SURFACE(3,2,((#206786,#206787,#206788),(#206789,#206790,#206791),
(#206792,#206793,#206794),(#206795,#206796,#206797),(#206798,#206799,#206800),
(#206801,#206802,#206803)),.UNSPECIFIED.,.F.,.F.,.F.)
B_SPLINE_SURFACE_WITH_KNOTS((4,2,4),(3,3),(0.,0.000256592814262155,0.00051318562852431),
(0.,1.),.UNSPECIFIED.)
GEOMETRIC_REPRESENTATION_ITEM()
RATIONAL_B_SPLINE_SURFACE(((1.,0.708712527163649,1.),(1.,0.753780902613242,
1.),(1.,0.794538995769662,1.),(1.,0.855070770330658,1.),(1.,0.875018427445663,
1.),(1.,0.874619707139383,1.)))
REPRESENTATION_ITEM('')
SURFACE()
);
#3017=(
BOUNDED_SURFACE()
B_SPLINE_SURFACE(3,2,((#206805,#206806,#206807),(#206808,#206809,#206810),
(#206811,#206812,#206813),(#206814,#206815,#206816)),.UNSPECIFIED.,.F.,
 .F.,.F.)
B_SPLINE_SURFACE_WITH_KNOTS((4,4),(3,3),(2.71050543121376E-20,0.0005118150724304),
(0.,1.00105598365872),.UNSPECIFIED.)
GEOMETRIC_REPRESENTATION_ITEM()
RATIONAL_B_SPLINE_SURFACE(((1.,0.70679749073373,1.00061923411696),(1.,0.706182062146616,
1.00062053388202),(1.,0.705584062769036,1.00062179683717),(1.,0.705266224770467,
1.00062246810063)))
REPRESENTATION_ITEM('')
SURFACE()
);
#3018=(
BOUNDED_SURFACE()
B_SPLINE_SURFACE(3,2,((#206822,#206823,#206824),(#206825,#206826,#206827),
(#206828,#206829,#206830),(#206831,#206832,#206833),(#206834,#206835,#206836),
(#206837,#206838,#206839)),.UNSPECIFIED.,.F.,.F.,.F.)
B_SPLINE_SURFACE_WITH_KNOTS((4,2,4),(3,3),(-3.15773882736403E-18,0.000257652232350885,
0.000515304464701772),(0.,1.),.UNSPECIFIED.)
GEOMETRIC_REPRESENTATION_ITEM()
RATIONAL_B_SPLINE_SURFACE(((1.,0.874619707139379,1.),(1.,0.874861180430934,
1.),(1.,0.855455725920527,1.),(1.,0.794699358955577,1.),(1.,0.753768977788386,
1.),(1.,0.708712527163667,1.)))
REPRESENTATION_ITEM('')
SURFACE()
);
#3019=(
BOUNDED_SURFACE()
B_SPLINE_SURFACE(3,2,((#206845,#206846,#206847),(#206848,#206849,#206850),
(#206851,#206852,#206853),(#206854,#206855,#206856)),.UNSPECIFIED.,.F.,
 .F.,.F.)
B_SPLINE_SURFACE_WITH_KNOTS((4,4),(3,3),(0.,0.000397394373651917),(0.,1.),
 .UNSPECIFIED.)
GEOMETRIC_REPRESENTATION_ITEM()
RATIONAL_B_SPLINE_SURFACE(((1.,0.707106781186553,1.),(1.,0.707752587915892,
1.),(1.,0.708377654540686,1.),(1.,0.708689770883343,1.)))
REPRESENTATION_ITEM('')
SURFACE()
);
#3020=(
BOUNDED_SURFACE()
B_SPLINE_SURFACE(3,2,((#206858,#206859,#206860),(#206861,#206862,#206863),
(#206864,#206865,#206866),(#206867,#206868,#206869)),.UNSPECIFIED.,.F.,
 .F.,.F.)
B_SPLINE_SURFACE_WITH_KNOTS((4,4),(3,3),(0.,0.000511815456479782),(0.,1.00105873160063),
 .UNSPECIFIED.)
GEOMETRIC_REPRESENTATION_ITEM()
RATIONAL_B_SPLINE_SURFACE(((1.,0.708394529056139,1.00061746385401),(1.,
0.708058564166688,1.0006181752473),(1.,0.707430835371857,1.00061950443992),
(1.,0.70679668588018,1.00062084722814)))
REPRESENTATION_ITEM('')
SURFACE()
);
#3021=(
BOUNDED_SURFACE()
B_SPLINE_SURFACE(3,2,((#206875,#206876,#206877),(#206878,#206879,#206880),
(#206881,#206882,#206883),(#206884,#206885,#206886)),.UNSPECIFIED.,.F.,
 .F.,.F.)
B_SPLINE_SURFACE_WITH_KNOTS((4,4),(3,3),(0.,0.000397394465448316),(0.,1.),
 .UNSPECIFIED.)
GEOMETRIC_REPRESENTATION_ITEM()
RATIONAL_B_SPLINE_SURFACE(((1.,0.705498956110747,1.),(1.,0.705821764811782,
1.),(1.,0.706461952521135,1.),(1.,0.707106781186548,1.)))
REPRESENTATION_ITEM('')
SURFACE()
);
#3022=(
BOUNDED_SURFACE()
B_SPLINE_SURFACE(3,2,((#206892,#206893,#206894),(#206895,#206896,#206897),
(#206898,#206899,#206900),(#206901,#206902,#206903)),.UNSPECIFIED.,.F.,
 .F.,.F.)
B_SPLINE_SURFACE_WITH_KNOTS((4,4),(3,3),(0.,0.000397394410828751),(0.,1.),
 .UNSPECIFIED.)
GEOMETRIC_REPRESENTATION_ITEM()
RATIONAL_B_SPLINE_SURFACE(((1.,0.708689770883333,1.),(1.,0.708376440034456,
1.),(1.,0.707750498698422,1.),(1.,0.707106781186552,1.)))
REPRESENTATION_ITEM('')
SURFACE()
);
#3023=(
BOUNDED_SURFACE()
B_SPLINE_SURFACE(3,2,((#206909,#206910,#206911),(#206912,#206913,#206914),
(#206915,#206916,#206917),(#206918,#206919,#206920)),.UNSPECIFIED.,.F.,
 .F.,.F.)
B_SPLINE_SURFACE_WITH_KNOTS((4,4),(3,3),(0.,0.000511815090126177),(0.,1.00105592270027),
 .UNSPECIFIED.)
GEOMETRIC_REPRESENTATION_ITEM()
RATIONAL_B_SPLINE_SURFACE(((1.,0.70526624271804,1.0006224321297),(1.,0.70558408590973,
1.00062176089402),(1.,0.706182089451049,1.00062049800299),(1.,0.706797508588047,
1.00061919833292)))
REPRESENTATION_ITEM('')
SURFACE()
);
#3024=(
BOUNDED_SURFACE()
B_SPLINE_SURFACE(3,2,((#206922,#206923,#206924),(#206925,#206926,#206927),
(#206928,#206929,#206930),(#206931,#206932,#206933)),.UNSPECIFIED.,.F.,
 .F.,.F.)
B_SPLINE_SURFACE_WITH_KNOTS((4,4),(3,3),(-7.04731412115578E-18,0.000397394428086623),
(0.,1.),.UNSPECIFIED.)
GEOMETRIC_REPRESENTATION_ITEM()
RATIONAL_B_SPLINE_SURFACE(((1.,0.707106781186552,1.),(1.,0.706459846759081,
1.),(1.,0.705820510737286,1.),(1.,0.705498956110751,1.)))
REPRESENTATION_ITEM('')
SURFACE()
);
#3025=(
BOUNDED_SURFACE()
B_SPLINE_SURFACE(3,2,((#206939,#206940,#206941),(#206942,#206943,#206944),
(#206945,#206946,#206947),(#206948,#206949,#206950),(#206951,#206952,#206953),
(#206954,#206955,#206956)),.UNSPECIFIED.,.F.,.F.,.F.)
B_SPLINE_SURFACE_WITH_KNOTS((4,2,4),(3,3),(0.,0.000257953807872837,0.000515907615745674),
(0.,1.),.UNSPECIFIED.)
GEOMETRIC_REPRESENTATION_ITEM()
RATIONAL_B_SPLINE_SURFACE(((1.,0.874619707139392,1.),(1.,0.874834349678964,
1.),(1.,0.854686104157824,1.),(1.,0.792476597915125,1.),(1.,0.750887854595146,
1.),(1.,0.705585838031451,1.)))
REPRESENTATION_ITEM('')
SURFACE()
);
#3026=(
BOUNDED_SURFACE()
B_SPLINE_SURFACE(3,2,((#206962,#206963,#206964),(#206965,#206966,#206967),
(#206968,#206969,#206970),(#206971,#206972,#206973)),.UNSPECIFIED.,.F.,
 .F.,.F.)
B_SPLINE_SURFACE_WITH_KNOTS((4,4),(3,3),(0.,0.000511815437699147),(0.,1.00105881331747),
 .UNSPECIFIED.)
GEOMETRIC_REPRESENTATION_ITEM()
RATIONAL_B_SPLINE_SURFACE(((1.,0.706796661945872,1.00062089519812),(1.,
0.707430821224739,1.00061955228554),(1.,0.708058545830266,1.00061822299919),
(1.,0.708394505252261,1.00061751156257)))
REPRESENTATION_ITEM('')
SURFACE()
);
#3027=(
BOUNDED_SURFACE()
B_SPLINE_SURFACE(3,2,((#206975,#206976,#206977),(#206978,#206979,#206980),
(#206981,#206982,#206983),(#206984,#206985,#206986),(#206987,#206988,#206989),
(#206990,#206991,#206992)),.UNSPECIFIED.,.F.,.F.,.F.)
B_SPLINE_SURFACE_WITH_KNOTS((4,2,4),(3,3),(0.,0.00025691531753126,0.000513830635062519),
(0.,1.),.UNSPECIFIED.)
GEOMETRIC_REPRESENTATION_ITEM()
RATIONAL_B_SPLINE_SURFACE(((1.,0.705585838031444,1.),(1.,0.750902433543079,
1.),(1.,0.79232953008207,1.),(1.,0.854288401594637,1.),(1.,0.874998031124809,
1.),(1.,0.874619707139393,1.)))
REPRESENTATION_ITEM('')
SURFACE()
);
#3028=(
BOUNDED_SURFACE()
B_SPLINE_SURFACE(3,2,((#206998,#206999,#207000),(#207001,#207002,#207003),
(#207004,#207005,#207006),(#207007,#207008,#207009),(#207010,#207011,#207012),
(#207013,#207014,#207015)),.UNSPECIFIED.,.F.,.F.,.F.)
B_SPLINE_SURFACE_WITH_KNOTS((4,2,4),(3,3),(0.,0.000256592814262157,0.000513185628524314),
(0.,1.),.UNSPECIFIED.)
GEOMETRIC_REPRESENTATION_ITEM()
RATIONAL_B_SPLINE_SURFACE(((1.,0.708712527163661,1.),(1.,0.753780902613635,
1.),(1.,0.794538995769146,1.),(1.,0.855070770331154,1.),(1.,0.875018427445277,
1.),(1.,0.874619707139389,1.)))
REPRESENTATION_ITEM('')
SURFACE()
);
#3029=(
BOUNDED_SURFACE()
B_SPLINE_SURFACE(3,2,((#207017,#207018,#207019),(#207020,#207021,#207022),
(#207023,#207024,#207025),(#207026,#207027,#207028)),.UNSPECIFIED.,.F.,
 .F.,.F.)
B_SPLINE_SURFACE_WITH_KNOTS((4,4),(3,3),(2.71050543121376E-20,0.000511815072430401),
(0.,1.00105598365816),.UNSPECIFIED.)
GEOMETRIC_REPRESENTATION_ITEM()
RATIONAL_B_SPLINE_SURFACE(((1.,0.706797490733895,1.00061923411663),(1.,
0.706182062146812,1.00062053388169),(1.,0.705584062769175,1.00062179683683),
(1.,0.705266224770663,1.0006224681003)))
REPRESENTATION_ITEM('')
SURFACE()
);
#3030=(
BOUNDED_SURFACE()
B_SPLINE_SURFACE(3,2,((#207034,#207035,#207036),(#207037,#207038,#207039),
(#207040,#207041,#207042),(#207043,#207044,#207045),(#207046,#207047,#207048),
(#207049,#207050,#207051)),.UNSPECIFIED.,.F.,.F.,.F.)
B_SPLINE_SURFACE_WITH_KNOTS((4,2,4),(3,3),(-1.35525271560688E-20,0.000257652232350881,
0.000515304464701761),(0.,1.),.UNSPECIFIED.)
GEOMETRIC_REPRESENTATION_ITEM()
RATIONAL_B_SPLINE_SURFACE(((1.,0.874619707139399,1.),(1.,0.87486118043092,
1.),(1.,0.855455725920554,1.),(1.,0.794699358955568,1.),(1.,0.753768977788393,
1.),(1.,0.708712527163671,1.)))
REPRESENTATION_ITEM('')
SURFACE()
);
#3031=(
BOUNDED_SURFACE()
B_SPLINE_SURFACE(3,2,((#207057,#207058,#207059),(#207060,#207061,#207062),
(#207063,#207064,#207065),(#207066,#207067,#207068)),.UNSPECIFIED.,.F.,
 .F.,.F.)
B_SPLINE_SURFACE_WITH_KNOTS((4,4),(3,3),(0.,0.000397394373651918),(0.,1.),
 .UNSPECIFIED.)
GEOMETRIC_REPRESENTATION_ITEM()
RATIONAL_B_SPLINE_SURFACE(((1.,0.707106781186552,1.),(1.,0.707752587915896,
1.),(1.,0.708377654540672,1.),(1.,0.708689770883335,1.)))
REPRESENTATION_ITEM('')
SURFACE()
);
#3032=(
BOUNDED_SURFACE()
B_SPLINE_SURFACE(3,2,((#207070,#207071,#207072),(#207073,#207074,#207075),
(#207076,#207077,#207078),(#207079,#207080,#207081)),.UNSPECIFIED.,.F.,
 .F.,.F.)
B_SPLINE_SURFACE_WITH_KNOTS((4,4),(3,3),(0.,0.000511815456479794),(0.,1.00105873159933),
 .UNSPECIFIED.)
GEOMETRIC_REPRESENTATION_ITEM()
RATIONAL_B_SPLINE_SURFACE(((1.,0.708394529056518,1.00061746385325),(1.,
0.708058564167052,1.00061817524654),(1.,0.707430835372237,1.00061950443916),
(1.,0.706796685880559,1.00062084722737)))
REPRESENTATION_ITEM('')
SURFACE()
);
#3033=(
BOUNDED_SURFACE()
B_SPLINE_SURFACE(3,2,((#207087,#207088,#207089),(#207090,#207091,#207092),
(#207093,#207094,#207095),(#207096,#207097,#207098)),.UNSPECIFIED.,.F.,
 .F.,.F.)
B_SPLINE_SURFACE_WITH_KNOTS((4,4),(3,3),(0.,0.000397394465448303),(0.,1.),
 .UNSPECIFIED.)
GEOMETRIC_REPRESENTATION_ITEM()
RATIONAL_B_SPLINE_SURFACE(((1.,0.705498956110754,1.),(1.,0.705821764811766,
1.),(1.,0.706461952521146,1.),(1.,0.707106781186548,1.)))
REPRESENTATION_ITEM('')
SURFACE()
);
#3034=(
BOUNDED_SURFACE()
B_SPLINE_SURFACE(3,2,((#207104,#207105,#207106),(#207107,#207108,#207109),
(#207110,#207111,#207112),(#207113,#207114,#207115)),.UNSPECIFIED.,.F.,
 .F.,.F.)
B_SPLINE_SURFACE_WITH_KNOTS((4,4),(3,3),(0.,0.000397394410828732),(0.,1.),
 .UNSPECIFIED.)
GEOMETRIC_REPRESENTATION_ITEM()
RATIONAL_B_SPLINE_SURFACE(((1.,0.708689770883346,1.),(1.,0.708376440034465,
1.),(1.,0.707750498698423,1.),(1.,0.707106781186548,1.)))
REPRESENTATION_ITEM('')
SURFACE()
);
#3035=(
BOUNDED_SURFACE()
B_SPLINE_SURFACE(3,2,((#207121,#207122,#207123),(#207124,#207125,#207126),
(#207127,#207128,#207129),(#207130,#207131,#207132)),.UNSPECIFIED.,.F.,
 .F.,.F.)
B_SPLINE_SURFACE_WITH_KNOTS((4,4),(3,3),(0.,0.000511815090126172),(0.,1.00105592270163),
 .UNSPECIFIED.)
GEOMETRIC_REPRESENTATION_ITEM()
RATIONAL_B_SPLINE_SURFACE(((1.,0.705266242717656,1.0006224321305),(1.,0.705584085909297,
1.00062176089482),(1.,0.706182089450663,1.00062049800379),(1.,0.706797508587648,
1.00061919833372)))
REPRESENTATION_ITEM('')
SURFACE()
);
#3036=(
BOUNDED_SURFACE()
B_SPLINE_SURFACE(3,2,((#207134,#207135,#207136),(#207137,#207138,#207139),
(#207140,#207141,#207142),(#207143,#207144,#207145)),.UNSPECIFIED.,.F.,
 .F.,.F.)
B_SPLINE_SURFACE_WITH_KNOTS((4,4),(3,3),(0.,0.000397394428086631),(0.,1.),
 .UNSPECIFIED.)
GEOMETRIC_REPRESENTATION_ITEM()
RATIONAL_B_SPLINE_SURFACE(((1.,0.707106781186548,1.),(1.,0.706459846759101,
1.),(1.,0.705820510737274,1.),(1.,0.705498956110758,1.)))
REPRESENTATION_ITEM('')
SURFACE()
);
#3037=(
BOUNDED_SURFACE()
B_SPLINE_SURFACE(3,2,((#207151,#207152,#207153),(#207154,#207155,#207156),
(#207157,#207158,#207159),(#207160,#207161,#207162),(#207163,#207164,#207165),
(#207166,#207167,#207168)),.UNSPECIFIED.,.F.,.F.,.F.)
B_SPLINE_SURFACE_WITH_KNOTS((4,2,4),(3,3),(0.,0.000257953807872843,0.000515907615745686),
(0.,1.),.UNSPECIFIED.)
GEOMETRIC_REPRESENTATION_ITEM()
RATIONAL_B_SPLINE_SURFACE(((1.,0.874619707139387,1.),(1.,0.874834349679408,
1.),(1.,0.854686104157222,1.),(1.,0.792476597915714,1.),(1.,0.750887854594714,
1.),(1.,0.70558583803143,1.)))
REPRESENTATION_ITEM('')
SURFACE()
);
#3038=(
BOUNDED_SURFACE()
B_SPLINE_SURFACE(3,2,((#207174,#207175,#207176),(#207177,#207178,#207179),
(#207180,#207181,#207182),(#207183,#207184,#207185)),.UNSPECIFIED.,.F.,
 .F.,.F.)
B_SPLINE_SURFACE_WITH_KNOTS((4,4),(3,3),(0.,0.000511815437699148),(0.,1.00105881331484),
 .UNSPECIFIED.)
GEOMETRIC_REPRESENTATION_ITEM()
RATIONAL_B_SPLINE_SURFACE(((1.,0.706796661946642,1.00062089519658),(1.,
0.707430821225516,1.000619552284),(1.,0.708058545831031,1.00061822299766),
(1.,0.708394505253015,1.00061751156104)))
REPRESENTATION_ITEM('')
SURFACE()
);
#3039=(
BOUNDED_SURFACE()
B_SPLINE_SURFACE(3,2,((#207187,#207188,#207189),(#207190,#207191,#207192),
(#207193,#207194,#207195),(#207196,#207197,#207198),(#207199,#207200,#207201),
(#207202,#207203,#207204)),.UNSPECIFIED.,.F.,.F.,.F.)
B_SPLINE_SURFACE_WITH_KNOTS((4,2,4),(3,3),(2.71050543121376E-20,0.000256915317531269,
0.000513830635062539),(0.,1.),.UNSPECIFIED.)
GEOMETRIC_REPRESENTATION_ITEM()
RATIONAL_B_SPLINE_SURFACE(((1.,0.705585838031441,1.),(1.,0.750902433542262,
1.),(1.,0.792329530083195,1.),(1.,0.854288401593528,1.),(1.,0.874998031125646,
1.),(1.,0.874619707139414,1.)))
REPRESENTATION_ITEM('')
SURFACE()
);
#3040=(
BOUNDED_SURFACE()
B_SPLINE_SURFACE(3,2,((#207210,#207211,#207212),(#207213,#207214,#207215),
(#207216,#207217,#207218),(#207219,#207220,#207221),(#207222,#207223,#207224),
(#207225,#207226,#207227)),.UNSPECIFIED.,.F.,.F.,.F.)
B_SPLINE_SURFACE_WITH_KNOTS((4,2,4),(3,3),(-9.64939933512099E-18,0.00025659281426215,
0.000513185628524309),(0.,1.),.UNSPECIFIED.)
GEOMETRIC_REPRESENTATION_ITEM()
RATIONAL_B_SPLINE_SURFACE(((1.,0.708712527163639,1.),(1.,0.753780902613581,
1.),(1.,0.79453899576923,1.),(1.,0.855070770331076,1.),(1.,0.875018427445352,
1.),(1.,0.874619707139392,1.)))
REPRESENTATION_ITEM('')
SURFACE()
);
#3041=(
BOUNDED_SURFACE()
B_SPLINE_SURFACE(3,2,((#207229,#207230,#207231),(#207232,#207233,#207234),
(#207235,#207236,#207237),(#207238,#207239,#207240)),.UNSPECIFIED.,.F.,
 .F.,.F.)
B_SPLINE_SURFACE_WITH_KNOTS((4,4),(3,3),(0.,0.000511815072430398),(0.,1.00105598365608),
 .UNSPECIFIED.)
GEOMETRIC_REPRESENTATION_ITEM()
RATIONAL_B_SPLINE_SURFACE(((1.,0.706797490734501,1.00061923411541),(1.,
0.706182062147433,1.00062053388047),(1.,0.705584062769772,1.00062179683561),
(1.,0.705266224771265,1.00062246809907)))
REPRESENTATION_ITEM('')
SURFACE()
);
#3042=(
BOUNDED_SURFACE()
B_SPLINE_SURFACE(3,2,((#207246,#207247,#207248),(#207249,#207250,#207251),
(#207252,#207253,#207254),(#207255,#207256,#207257),(#207258,#207259,#207260),
(#207261,#207262,#207263)),.UNSPECIFIED.,.F.,.F.,.F.)
B_SPLINE_SURFACE_WITH_KNOTS((4,2,4),(3,3),(-8.53809210832335E-19,0.000257652232350883,
0.000515304464701767),(0.,1.),.UNSPECIFIED.)
GEOMETRIC_REPRESENTATION_ITEM()
RATIONAL_B_SPLINE_SURFACE(((1.,0.874619707139377,1.),(1.,0.874861180430964,
1.),(1.,0.855455725920508,1.),(1.,0.794699358955598,1.),(1.,0.753768977788379,
1.),(1.,0.708712527163652,1.)))
REPRESENTATION_ITEM('')
SURFACE()
);
#3043=(
BOUNDED_SURFACE()
B_SPLINE_SURFACE(3,2,((#207269,#207270,#207271),(#207272,#207273,#207274),
(#207275,#207276,#207277),(#207278,#207279,#207280)),.UNSPECIFIED.,.F.,
 .F.,.F.)
B_SPLINE_SURFACE_WITH_KNOTS((4,4),(3,3),(0.,0.000397394373651916),(0.,1.),
 .UNSPECIFIED.)
GEOMETRIC_REPRESENTATION_ITEM()
RATIONAL_B_SPLINE_SURFACE(((1.,0.707106781186548,1.),(1.,0.707752587915897,
1.),(1.,0.708377654540682,1.),(1.,0.708689770883335,1.)))
REPRESENTATION_ITEM('')
SURFACE()
);
#3044=(
BOUNDED_SURFACE()
B_SPLINE_SURFACE(3,2,((#207282,#207283,#207284),(#207285,#207286,#207287),
(#207288,#207289,#207290),(#207291,#207292,#207293)),.UNSPECIFIED.,.F.,
 .F.,.F.)
B_SPLINE_SURFACE_WITH_KNOTS((4,4),(3,3),(0.,0.000511815456479795),(0.,1.00105873160039),
 .UNSPECIFIED.)
GEOMETRIC_REPRESENTATION_ITEM()
RATIONAL_B_SPLINE_SURFACE(((1.,0.708394529056206,1.00061746385387),(1.,
0.708058564166753,1.00061817524716),(1.,0.70743083537193,1.00061950443978),
(1.,0.706796685880251,1.00062084722799)))
REPRESENTATION_ITEM('')
SURFACE()
);
#3045=(
BOUNDED_SURFACE()
B_SPLINE_SURFACE(3,2,((#207299,#207300,#207301),(#207302,#207303,#207304),
(#207305,#207306,#207307),(#207308,#207309,#207310)),.UNSPECIFIED.,.F.,
 .F.,.F.)
B_SPLINE_SURFACE_WITH_KNOTS((4,4),(3,3),(-6.50521303491303E-18,0.000397394465448295),
(0.,1.),.UNSPECIFIED.)
GEOMETRIC_REPRESENTATION_ITEM()
RATIONAL_B_SPLINE_SURFACE(((1.,0.705498956110765,1.),(1.,0.705821764811772,
1.),(1.,0.706461952521134,1.),(1.,0.70710678118655,1.)))
REPRESENTATION_ITEM('')
SURFACE()
);
#3046=(
BOUNDED_SURFACE()
B_SPLINE_SURFACE(3,2,((#207316,#207317,#207318),(#207319,#207320,#207321),
(#207322,#207323,#207324),(#207325,#207326,#207327)),.UNSPECIFIED.,.F.,
 .F.,.F.)
B_SPLINE_SURFACE_WITH_KNOTS((4,4),(3,3),(0.,0.000397394410828733),(0.,1.),
 .UNSPECIFIED.)
GEOMETRIC_REPRESENTATION_ITEM()
RATIONAL_B_SPLINE_SURFACE(((1.,0.708689770883334,1.),(1.,0.708376440034491,
1.),(1.,0.707750498698413,1.),(1.,0.707106781186548,1.)))
REPRESENTATION_ITEM('')
SURFACE()
);
#3047=(
BOUNDED_SURFACE()
B_SPLINE_SURFACE(3,2,((#207333,#207334,#207335),(#207336,#207337,#207338),
(#207339,#207340,#207341),(#207342,#207343,#207344)),.UNSPECIFIED.,.F.,
 .F.,.F.)
B_SPLINE_SURFACE_WITH_KNOTS((4,4),(3,3),(0.,0.000511815090126173),(0.,1.00105592270208),
 .UNSPECIFIED.)
GEOMETRIC_REPRESENTATION_ITEM()
RATIONAL_B_SPLINE_SURFACE(((1.,0.705266242717518,1.00062243213077),(1.,
0.705584085909175,1.00062176089508),(1.,0.706182089450533,1.00062049800405),
(1.,0.706797508587518,1.00061919833398)))
REPRESENTATION_ITEM('')
SURFACE()
);
#3048=(
BOUNDED_SURFACE()
B_SPLINE_SURFACE(3,2,((#207346,#207347,#207348),(#207349,#207350,#207351),
(#207352,#207353,#207354),(#207355,#207356,#207357)),.UNSPECIFIED.,.F.,
 .F.,.F.)
B_SPLINE_SURFACE_WITH_KNOTS((4,4),(3,3),(0.,0.000397394428086626),(0.,1.),
 .UNSPECIFIED.)
GEOMETRIC_REPRESENTATION_ITEM()
RATIONAL_B_SPLINE_SURFACE(((1.,0.707106781186548,1.),(1.,0.7064598467591,
1.),(1.,0.70582051073725,1.),(1.,0.705498956110749,1.)))
REPRESENTATION_ITEM('')
SURFACE()
);
#3049=(
BOUNDED_SURFACE()
B_SPLINE_SURFACE(3,2,((#207363,#207364,#207365),(#207366,#207367,#207368),
(#207369,#207370,#207371),(#207372,#207373,#207374),(#207375,#207376,#207377),
(#207378,#207379,#207380)),.UNSPECIFIED.,.F.,.F.,.F.)
B_SPLINE_SURFACE_WITH_KNOTS((4,2,4),(3,3),(0.,0.000257953807872854,0.000515907615745708),
(0.,1.),.UNSPECIFIED.)
GEOMETRIC_REPRESENTATION_ITEM()
RATIONAL_B_SPLINE_SURFACE(((1.,0.874619707139392,1.),(1.,0.874834349678953,
1.),(1.,0.854686104157836,1.),(1.,0.792476597915084,1.),(1.,0.750887854595165,
1.),(1.,0.705585838031428,1.)))
REPRESENTATION_ITEM('')
SURFACE()
);
#3050=(
BOUNDED_SURFACE()
B_SPLINE_SURFACE(3,2,((#207383,#207384,#207385),(#207386,#207387,#207388),
(#207389,#207390,#207391),(#207392,#207393,#207394)),.UNSPECIFIED.,.F.,
 .F.,.F.)
B_SPLINE_SURFACE_WITH_KNOTS((4,4),(3,3),(0.,0.000511815437699152),(0.,1.0010588133155),
 .UNSPECIFIED.)
GEOMETRIC_REPRESENTATION_ITEM()
RATIONAL_B_SPLINE_SURFACE(((1.,0.706796661946447,1.00062089519696),(1.,
0.707430821225326,1.00061955228439),(1.,0.708058545830837,1.00061822299804),
(1.,0.708394505252831,1.00061751156143)))
REPRESENTATION_ITEM('')
SURFACE()
);
#3051=(
BOUNDED_SURFACE()
B_SPLINE_SURFACE(3,2,((#207396,#207397,#207398),(#207399,#207400,#207401),
(#207402,#207403,#207404),(#207405,#207406,#207407),(#207408,#207409,#207410),
(#207411,#207412,#207413)),.UNSPECIFIED.,.F.,.F.,.F.)
B_SPLINE_SURFACE_WITH_KNOTS((4,2,4),(3,3),(0.,0.000256915317531263,0.000513830635062526),
(0.,1.),.UNSPECIFIED.)
GEOMETRIC_REPRESENTATION_ITEM()
RATIONAL_B_SPLINE_SURFACE(((1.,0.705585838031434,1.),(1.,0.750902433542931,
1.),(1.,0.792329530082276,1.),(1.,0.854288401594432,1.),(1.,0.874998031124954,
1.),(1.,0.874619707139392,1.)))
REPRESENTATION_ITEM('')
SURFACE()
);
#3052=(
BOUNDED_SURFACE()
B_SPLINE_SURFACE(3,2,((#207419,#207420,#207421),(#207422,#207423,#207424),
(#207425,#207426,#207427),(#207428,#207429,#207430),(#207431,#207432,#207433),
(#207434,#207435,#207436)),.UNSPECIFIED.,.F.,.F.,.F.)
B_SPLINE_SURFACE_WITH_KNOTS((4,2,4),(3,3),(-9.7307144980574E-18,0.000256592814262151,
0.000513185628524313),(0.,1.),.UNSPECIFIED.)
GEOMETRIC_REPRESENTATION_ITEM()
RATIONAL_B_SPLINE_SURFACE(((1.,0.708712527163666,1.),(1.,0.753780902613597,
1.),(1.,0.794538995769187,1.),(1.,0.855070770331129,1.),(1.,0.875018427445299,
1.),(1.,0.87461970713939,1.)))
REPRESENTATION_ITEM('')
SURFACE()
);
#3053=(
BOUNDED_SURFACE()
B_SPLINE_SURFACE(3,2,((#207437,#207438,#207439),(#207440,#207441,#207442),
(#207443,#207444,#207445),(#207446,#207447,#207448)),.UNSPECIFIED.,.F.,
 .F.,.F.)
B_SPLINE_SURFACE_WITH_KNOTS((4,4),(3,3),(0.,0.000511815072430396),(0.,1.00105598365805),
 .UNSPECIFIED.)
GEOMETRIC_REPRESENTATION_ITEM()
RATIONAL_B_SPLINE_SURFACE(((1.,0.706797490733928,1.00061923411657),(1.,
0.706182062146832,1.00062053388163),(1.,0.705584062769228,1.00062179683677),
(1.,0.705266224770693,1.00062246810023)))
REPRESENTATION_ITEM('')
SURFACE()
);
#3054=(
BOUNDED_SURFACE()
B_SPLINE_SURFACE(3,2,((#207452,#207453,#207454),(#207455,#207456,#207457),
(#207458,#207459,#207460),(#207461,#207462,#207463),(#207464,#207465,#207466),
(#207467,#207468,#207469)),.UNSPECIFIED.,.F.,.F.,.F.)
B_SPLINE_SURFACE_WITH_KNOTS((4,2,4),(3,3),(-6.36968776335234E-19,0.000257652232350878,
0.000515304464701757),(0.,1.),.UNSPECIFIED.)
GEOMETRIC_REPRESENTATION_ITEM()
RATIONAL_B_SPLINE_SURFACE(((1.,0.874619707139396,1.),(1.,0.874861180430738,
1.),(1.,0.855455725920818,1.),(1.,0.794699358955304,1.),(1.,0.753768977788614,
1.),(1.,0.70871252716366,1.)))
REPRESENTATION_ITEM('')
SURFACE()
);
#3055=(
BOUNDED_SURFACE()
B_SPLINE_SURFACE(3,2,((#207475,#207476,#207477),(#207478,#207479,#207480),
(#207481,#207482,#207483),(#207484,#207485,#207486)),.UNSPECIFIED.,.F.,
 .F.,.F.)
B_SPLINE_SURFACE_WITH_KNOTS((4,4),(3,3),(0.,0.000397394373651917),(0.,1.),
 .UNSPECIFIED.)
GEOMETRIC_REPRESENTATION_ITEM()
RATIONAL_B_SPLINE_SURFACE(((1.,0.707106781186548,1.),(1.,0.70775258791587,
1.),(1.,0.708377654540715,1.),(1.,0.708689770883311,1.)))
REPRESENTATION_ITEM('')
SURFACE()
);
#3056=(
BOUNDED_SURFACE()
B_SPLINE_SURFACE(3,2,((#207488,#207489,#207490),(#207491,#207492,#207493),
(#207494,#207495,#207496),(#207497,#207498,#207499)),.UNSPECIFIED.,.F.,
 .F.,.F.)
B_SPLINE_SURFACE_WITH_KNOTS((4,4),(3,3),(-6.42389787197661E-18,0.000511815456479785),
(0.,1.00105873159879),.UNSPECIFIED.)
GEOMETRIC_REPRESENTATION_ITEM()
RATIONAL_B_SPLINE_SURFACE(((1.,0.708394529056662,1.00061746385294),(1.,
0.708058564167226,1.00061817524623),(1.,0.707430835372388,1.00061950443885),
(1.,0.706796685880717,1.00062084722706)))
REPRESENTATION_ITEM('')
SURFACE()
);
#3057=(
BOUNDED_SURFACE()
B_SPLINE_SURFACE(3,2,((#207505,#207506,#207507),(#207508,#207509,#207510),
(#207511,#207512,#207513),(#207514,#207515,#207516)),.UNSPECIFIED.,.F.,
 .F.,.F.)
B_SPLINE_SURFACE_WITH_KNOTS((4,4),(3,3),(0.,0.000397394465448298),(0.,1.),
 .UNSPECIFIED.)
GEOMETRIC_REPRESENTATION_ITEM()
RATIONAL_B_SPLINE_SURFACE(((1.,0.705498956110772,1.),(1.,0.705821764811771,
1.),(1.,0.706461952521147,1.),(1.,0.707106781186547,1.)))
REPRESENTATION_ITEM('')
SURFACE()
);
#3058=(
BOUNDED_SURFACE()
B_SPLINE_SURFACE(3,2,((#207522,#207523,#207524),(#207525,#207526,#207527),
(#207528,#207529,#207530),(#207531,#207532,#207533)),.UNSPECIFIED.,.F.,
 .F.,.F.)
B_SPLINE_SURFACE_WITH_KNOTS((4,4),(3,3),(0.,0.000397394410828734),(0.,1.),
 .UNSPECIFIED.)
GEOMETRIC_REPRESENTATION_ITEM()
RATIONAL_B_SPLINE_SURFACE(((1.,0.708689770883325,1.),(1.,0.708376440034491,
1.),(1.,0.707750498698406,1.),(1.,0.707106781186545,1.)))
REPRESENTATION_ITEM('')
SURFACE()
);
#3059=(
BOUNDED_SURFACE()
B_SPLINE_SURFACE(3,2,((#207539,#207540,#207541),(#207542,#207543,#207544),
(#207545,#207546,#207547),(#207548,#207549,#207550)),.UNSPECIFIED.,.F.,
 .F.,.F.)
B_SPLINE_SURFACE_WITH_KNOTS((4,4),(3,3),(0.,0.000511815090126171),(0.,1.00105592270213),
 .UNSPECIFIED.)
GEOMETRIC_REPRESENTATION_ITEM()
RATIONAL_B_SPLINE_SURFACE(((1.,0.705266242717511,1.0006224321308),(1.,0.705584085909147,
1.00062176089511),(1.,0.706182089450526,1.00062049800408),(1.,0.706797508587502,
1.00061919833401)))
REPRESENTATION_ITEM('')
SURFACE()
);
#3060=(
BOUNDED_SURFACE()
B_SPLINE_SURFACE(3,2,((#207552,#207553,#207554),(#207555,#207556,#207557),
(#207558,#207559,#207560),(#207561,#207562,#207563)),.UNSPECIFIED.,.F.,
 .F.,.F.)
B_SPLINE_SURFACE_WITH_KNOTS((4,4),(3,3),(-6.88468379528295E-18,0.000397394428086618),
(0.,1.),.UNSPECIFIED.)
GEOMETRIC_REPRESENTATION_ITEM()
RATIONAL_B_SPLINE_SURFACE(((1.,0.707106781186545,1.),(1.,0.706459846759105,
1.),(1.,0.705820510737275,1.),(1.,0.705498956110758,1.)))
REPRESENTATION_ITEM('')
SURFACE()
);
#3061=(
BOUNDED_SURFACE()
B_SPLINE_SURFACE(3,2,((#207569,#207570,#207571),(#207572,#207573,#207574),
(#207575,#207576,#207577),(#207578,#207579,#207580),(#207581,#207582,#207583),
(#207584,#207585,#207586)),.UNSPECIFIED.,.F.,.F.,.F.)
B_SPLINE_SURFACE_WITH_KNOTS((4,2,4),(3,3),(-8.53809210832335E-19,0.000257953807872851,
0.000515907615745703),(0.,1.),.UNSPECIFIED.)
GEOMETRIC_REPRESENTATION_ITEM()
RATIONAL_B_SPLINE_SURFACE(((1.,0.874619707139387,1.),(1.,0.874834349679476,
1.),(1.,0.854686104157146,1.),(1.,0.792476597915799,1.),(1.,0.750887854594649,
1.),(1.,0.70558583803143,1.)))
REPRESENTATION_ITEM('')
SURFACE()
);
#3062=(
BOUNDED_SURFACE()
B_SPLINE_SURFACE(3,2,((#207592,#207593,#207594),(#207595,#207596,#207597),
(#207598,#207599,#207600),(#207601,#207602,#207603)),.UNSPECIFIED.,.F.,
 .F.,.F.)
B_SPLINE_SURFACE_WITH_KNOTS((4,4),(3,3),(0.,0.000511815437699152),(0.,1.00105881331394),
 .UNSPECIFIED.)
GEOMETRIC_REPRESENTATION_ITEM()
RATIONAL_B_SPLINE_SURFACE(((1.,0.706796661946908,1.00062089519604),(1.,
0.70743082122576,1.00061955228347),(1.,0.708058545831313,1.00061822299713),
(1.,0.708394505253263,1.00061751156051)))
REPRESENTATION_ITEM('')
SURFACE()
);
#3063=(
BOUNDED_SURFACE()
B_SPLINE_SURFACE(3,2,((#207605,#207606,#207607),(#207608,#207609,#207610),
(#207611,#207612,#207613),(#207614,#207615,#207616),(#207617,#207618,#207619),
(#207620,#207621,#207622)),.UNSPECIFIED.,.F.,.F.,.F.)
B_SPLINE_SURFACE_WITH_KNOTS((4,2,4),(3,3),(0.,0.000256915317531263,0.000513830635062525),
(0.,1.),.UNSPECIFIED.)
GEOMETRIC_REPRESENTATION_ITEM()
RATIONAL_B_SPLINE_SURFACE(((1.,0.705585838031452,1.),(1.,0.750902433542811,
1.),(1.,0.792329530082409,1.),(1.,0.854288401594288,1.),(1.,0.874998031125078,
1.),(1.,0.874619707139386,1.)))
REPRESENTATION_ITEM('')
SURFACE()
);
#3064=(
BOUNDED_SURFACE()
B_SPLINE_SURFACE(3,2,((#207628,#207629,#207630),(#207631,#207632,#207633),
(#207634,#207635,#207636),(#207637,#207638,#207639),(#207640,#207641,#207642),
(#207643,#207644,#207645)),.UNSPECIFIED.,.F.,.F.,.F.)
B_SPLINE_SURFACE_WITH_KNOTS((4,2,4),(3,3),(-1.0842021724855E-19,0.000256592814262156,
0.000513185628524312),(0.,1.),.UNSPECIFIED.)
GEOMETRIC_REPRESENTATION_ITEM()
RATIONAL_B_SPLINE_SURFACE(((1.,0.708712527163657,1.),(1.,0.753780902613831,
1.),(1.,0.794538995768884,1.),(1.,0.855070770331427,1.),(1.,0.875018427445074,
1.),(1.,0.874619707139396,1.)))
REPRESENTATION_ITEM('')
SURFACE()
);
#3065=(
BOUNDED_SURFACE()
B_SPLINE_SURFACE(3,2,((#207647,#207648,#207649),(#207650,#207651,#207652),
(#207653,#207654,#207655),(#207656,#207657,#207658)),.UNSPECIFIED.,.F.,
 .F.,.F.)
B_SPLINE_SURFACE_WITH_KNOTS((4,4),(3,3),(2.71050543121376E-20,0.000511815072430395),
(0.,1.00105598365712),.UNSPECIFIED.)
GEOMETRIC_REPRESENTATION_ITEM()
RATIONAL_B_SPLINE_SURFACE(((1.,0.706797490734199,1.00061923411602),(1.,
0.70618206214713,1.00062053388108),(1.,0.705584062769454,1.00062179683622),
(1.,0.705266224770955,1.00062246809969)))
REPRESENTATION_ITEM('')
SURFACE()
);
#3066=(
BOUNDED_SURFACE()
B_SPLINE_SURFACE(3,2,((#207664,#207665,#207666),(#207667,#207668,#207669),
(#207670,#207671,#207672),(#207673,#207674,#207675),(#207676,#207677,#207678),
(#207679,#207680,#207681)),.UNSPECIFIED.,.F.,.F.,.F.)
B_SPLINE_SURFACE_WITH_KNOTS((4,2,4),(3,3),(1.35525271560688E-20,0.000257652232350878,
0.000515304464701757),(0.,1.),.UNSPECIFIED.)
GEOMETRIC_REPRESENTATION_ITEM()
RATIONAL_B_SPLINE_SURFACE(((1.,0.874619707139391,1.),(1.,0.874861180431061,
1.),(1.,0.855455725920385,1.),(1.,0.794699358955754,1.),(1.,0.753768977788293,
1.),(1.,0.708712527163653,1.)))
REPRESENTATION_ITEM('')
SURFACE()
);
#3067=(
BOUNDED_SURFACE()
B_SPLINE_SURFACE(3,2,((#207687,#207688,#207689),(#207690,#207691,#207692),
(#207693,#207694,#207695),(#207696,#207697,#207698)),.UNSPECIFIED.,.F.,
 .F.,.F.)
B_SPLINE_SURFACE_WITH_KNOTS((4,4),(3,3),(0.,0.000397394373651917),(0.,1.),
 .UNSPECIFIED.)
GEOMETRIC_REPRESENTATION_ITEM()
RATIONAL_B_SPLINE_SURFACE(((1.,0.707106781186548,1.),(1.,0.707752587915895,
1.),(1.,0.708377654540701,1.),(1.,0.708689770883337,1.)))
REPRESENTATION_ITEM('')
SURFACE()
);
#3068=(
BOUNDED_SURFACE()
B_SPLINE_SURFACE(3,2,((#207700,#207701,#207702),(#207703,#207704,#207705),
(#207706,#207707,#207708),(#207709,#207710,#207711)),.UNSPECIFIED.,.F.,
 .F.,.F.)
B_SPLINE_SURFACE_WITH_KNOTS((4,4),(3,3),(0.,0.000511815456479796),(0.,1.00105873160039),
 .UNSPECIFIED.)
GEOMETRIC_REPRESENTATION_ITEM()
RATIONAL_B_SPLINE_SURFACE(((1.,0.708394529056226,1.00061746385387),(1.,
0.708058564166737,1.00061817524716),(1.,0.707430835371936,1.00061950443978),
(1.,0.70679668588025,1.00062084722799)))
REPRESENTATION_ITEM('')
SURFACE()
);
#3069=(
BOUNDED_SURFACE()
B_SPLINE_SURFACE(3,2,((#207717,#207718,#207719),(#207720,#207721,#207722),
(#207723,#207724,#207725),(#207726,#207727,#207728)),.UNSPECIFIED.,.F.,
 .F.,.F.)
B_SPLINE_SURFACE_WITH_KNOTS((4,4),(3,3),(-6.50521303491303E-18,0.000397394465448298),
(0.,1.),.UNSPECIFIED.)
GEOMETRIC_REPRESENTATION_ITEM()
RATIONAL_B_SPLINE_SURFACE(((1.,0.705498956110744,1.),(1.,0.705821764811786,
1.),(1.,0.706461952521138,1.),(1.,0.707106781186546,1.)))
REPRESENTATION_ITEM('')
SURFACE()
);
#3070=(
BOUNDED_SURFACE()
B_SPLINE_SURFACE(3,2,((#207734,#207735,#207736),(#207737,#207738,#207739),
(#207740,#207741,#207742),(#207743,#207744,#207745)),.UNSPECIFIED.,.F.,
 .F.,.F.)
B_SPLINE_SURFACE_WITH_KNOTS((4,4),(3,3),(0.,0.000397394410828756),(0.,1.),
 .UNSPECIFIED.)
GEOMETRIC_REPRESENTATION_ITEM()
RATIONAL_B_SPLINE_SURFACE(((1.,0.708689770883349,1.),(1.,0.708376440034465,
1.),(1.,0.707750498698429,1.),(1.,0.707106781186547,1.)))
REPRESENTATION_ITEM('')
SURFACE()
);
#3071=(
BOUNDED_SURFACE()
B_SPLINE_SURFACE(3,2,((#207751,#207752,#207753),(#207754,#207755,#207756),
(#207757,#207758,#207759),(#207760,#207761,#207762)),.UNSPECIFIED.,.F.,
 .F.,.F.)
B_SPLINE_SURFACE_WITH_KNOTS((4,4),(3,3),(0.,0.000511815090126185),(0.,1.00105592270233),
 .UNSPECIFIED.)
GEOMETRIC_REPRESENTATION_ITEM()
RATIONAL_B_SPLINE_SURFACE(((1.,0.705266242717445,1.00062243213092),(1.,
0.7055840859091,1.00062176089523),(1.,0.706182089450454,1.0006204980042),
(1.,0.706797508587444,1.00061919833413)))
REPRESENTATION_ITEM('')
SURFACE()
);
#3072=(
BOUNDED_SURFACE()
B_SPLINE_SURFACE(3,2,((#207764,#207765,#207766),(#207767,#207768,#207769),
(#207770,#207771,#207772),(#207773,#207774,#207775)),.UNSPECIFIED.,.F.,
 .F.,.F.)
B_SPLINE_SURFACE_WITH_KNOTS((4,4),(3,3),(0.,0.000397394428086631),(0.,1.),
 .UNSPECIFIED.)
GEOMETRIC_REPRESENTATION_ITEM()
RATIONAL_B_SPLINE_SURFACE(((1.,0.707106781186552,1.),(1.,0.706459846759088,
1.),(1.,0.705820510737275,1.),(1.,0.705498956110745,1.)))
REPRESENTATION_ITEM('')
SURFACE()
);
#3073=(
BOUNDED_SURFACE()
B_SPLINE_SURFACE(3,2,((#207781,#207782,#207783),(#207784,#207785,#207786),
(#207787,#207788,#207789),(#207790,#207791,#207792),(#207793,#207794,#207795),
(#207796,#207797,#207798)),.UNSPECIFIED.,.F.,.F.,.F.)
B_SPLINE_SURFACE_WITH_KNOTS((4,2,4),(3,3),(0.,0.000257953807872849,0.000515907615745697),
(0.,1.),.UNSPECIFIED.)
GEOMETRIC_REPRESENTATION_ITEM()
RATIONAL_B_SPLINE_SURFACE(((1.,0.874619707139393,1.),(1.,0.874834349679465,
1.),(1.,0.854686104157144,1.),(1.,0.792476597915797,1.),(1.,0.750887854594642,
1.),(1.,0.705585838031435,1.)))
REPRESENTATION_ITEM('')
SURFACE()
);
#3074=(
BOUNDED_SURFACE()
B_SPLINE_SURFACE(3,2,((#207804,#207805,#207806),(#207807,#207808,#207809),
(#207810,#207811,#207812),(#207813,#207814,#207815)),.UNSPECIFIED.,.F.,
 .F.,.F.)
B_SPLINE_SURFACE_WITH_KNOTS((4,4),(3,3),(0.,0.000511815437699151),(0.,1.00105881331716),
 .UNSPECIFIED.)
GEOMETRIC_REPRESENTATION_ITEM()
RATIONAL_B_SPLINE_SURFACE(((1.,0.706796661945962,1.00062089519794),(1.,
0.707430821224836,1.00061955228536),(1.,0.708058545830357,1.00061822299901),
(1.,0.70839450525234,1.00061751156239)))
REPRESENTATION_ITEM('')
SURFACE()
);
#3075=(
BOUNDED_SURFACE()
B_SPLINE_SURFACE(3,2,((#207817,#207818,#207819),(#207820,#207821,#207822),
(#207823,#207824,#207825),(#207826,#207827,#207828),(#207829,#207830,#207831),
(#207832,#207833,#207834)),.UNSPECIFIED.,.F.,.F.,.F.)
B_SPLINE_SURFACE_WITH_KNOTS((4,2,4),(3,3),(0.,0.000256915317531258,0.000513830635062516),
(0.,1.),.UNSPECIFIED.)
GEOMETRIC_REPRESENTATION_ITEM()
RATIONAL_B_SPLINE_SURFACE(((1.,0.705585838031428,1.),(1.,0.750902433542113,
1.),(1.,0.792329530083375,1.),(1.,0.854288401593323,1.),(1.,0.874998031125785,
1.),(1.,0.874619707139391,1.)))
REPRESENTATION_ITEM('')
SURFACE()
);
#3076=(
BOUNDED_SURFACE()
B_SPLINE_SURFACE(3,2,((#207840,#207841,#207842),(#207843,#207844,#207845),
(#207846,#207847,#207848),(#207849,#207850,#207851),(#207852,#207853,#207854),
(#207855,#207856,#207857)),.UNSPECIFIED.,.F.,.F.,.F.)
B_SPLINE_SURFACE_WITH_KNOTS((4,2,4),(3,3),(0.,0.000256592814262157,0.000513185628524314),
(0.,1.),.UNSPECIFIED.)
GEOMETRIC_REPRESENTATION_ITEM()
RATIONAL_B_SPLINE_SURFACE(((1.,0.708712527163666,1.),(1.,0.753780902613584,
1.),(1.,0.794538995769204,1.),(1.,0.855070770331107,1.),(1.,0.875018427445323,
1.),(1.,0.874619707139393,1.)))
REPRESENTATION_ITEM('')
SURFACE()
);
#3077=(
BOUNDED_SURFACE()
B_SPLINE_SURFACE(3,2,((#207859,#207860,#207861),(#207862,#207863,#207864),
(#207865,#207866,#207867),(#207868,#207869,#207870)),.UNSPECIFIED.,.F.,
 .F.,.F.)
B_SPLINE_SURFACE_WITH_KNOTS((4,4),(3,3),(2.71050543121376E-20,0.000511815072430406),
(0.,1.00105598365692),.UNSPECIFIED.)
GEOMETRIC_REPRESENTATION_ITEM()
RATIONAL_B_SPLINE_SURFACE(((1.,0.706797490734257,1.00061923411591),(1.,
0.706182062147172,1.00062053388097),(1.,0.705584062769546,1.0006217968361),
(1.,0.705266224771024,1.00062246809957)))
REPRESENTATION_ITEM('')
SURFACE()
);
#3078=(
BOUNDED_SURFACE()
B_SPLINE_SURFACE(3,2,((#207876,#207877,#207878),(#207879,#207880,#207881),
(#207882,#207883,#207884),(#207885,#207886,#207887),(#207888,#207889,#207890),
(#207891,#207892,#207893)),.UNSPECIFIED.,.F.,.F.,.F.)
B_SPLINE_SURFACE_WITH_KNOTS((4,2,4),(3,3),(-1.72117094882074E-18,0.000257652232350877,
0.000515304464701755),(0.,1.),.UNSPECIFIED.)
GEOMETRIC_REPRESENTATION_ITEM()
RATIONAL_B_SPLINE_SURFACE(((1.,0.874619707139395,1.),(1.,0.874861180430836,
1.),(1.,0.855455725920695,1.),(1.,0.794699358955469,1.),(1.,0.753768977788511,
1.),(1.,0.708712527163661,1.)))
REPRESENTATION_ITEM('')
SURFACE()
);
#3079=(
BOUNDED_SURFACE()
B_SPLINE_SURFACE(3,2,((#207899,#207900,#207901),(#207902,#207903,#207904),
(#207905,#207906,#207907),(#207908,#207909,#207910)),.UNSPECIFIED.,.F.,
 .F.,.F.)
B_SPLINE_SURFACE_WITH_KNOTS((4,4),(3,3),(0.,0.000397394373651921),(0.,1.),
 .UNSPECIFIED.)
GEOMETRIC_REPRESENTATION_ITEM()
RATIONAL_B_SPLINE_SURFACE(((1.,0.707106781186548,1.),(1.,0.707752587915898,
1.),(1.,0.70837765454066,1.),(1.,0.708689770883349,1.)))
REPRESENTATION_ITEM('')
SURFACE()
);
#3080=(
BOUNDED_SURFACE()
B_SPLINE_SURFACE(3,2,((#207912,#207913,#207914),(#207915,#207916,#207917),
(#207918,#207919,#207920),(#207921,#207922,#207923)),.UNSPECIFIED.,.F.,
 .F.,.F.)
B_SPLINE_SURFACE_WITH_KNOTS((4,4),(3,3),(-6.39679281766448E-18,0.000511815456479792),
(0.,1.00105873159887),.UNSPECIFIED.)
GEOMETRIC_REPRESENTATION_ITEM()
RATIONAL_B_SPLINE_SURFACE(((1.,0.70839452905664,1.00061746385298),(1.,0.708058564167196,
1.00061817524627),(1.,0.707430835372364,1.00061950443889),(1.,0.706796685880695,
1.0006208472271)))
REPRESENTATION_ITEM('')
SURFACE()
);
#3081=(
BOUNDED_SURFACE()
B_SPLINE_SURFACE(3,2,((#207929,#207930,#207931),(#207932,#207933,#207934),
(#207935,#207936,#207937),(#207938,#207939,#207940)),.UNSPECIFIED.,.F.,
 .F.,.F.)
B_SPLINE_SURFACE_WITH_KNOTS((4,4),(3,3),(0.,0.000397394465448321),(0.,1.),
 .UNSPECIFIED.)
GEOMETRIC_REPRESENTATION_ITEM()
RATIONAL_B_SPLINE_SURFACE(((1.,0.70549895611076,1.),(1.,0.705821764811783,
1.),(1.,0.706461952521143,1.),(1.,0.707106781186552,1.)))
REPRESENTATION_ITEM('')
SURFACE()
);
#3082=(
BOUNDED_SURFACE()
B_SPLINE_SURFACE(3,2,((#207946,#207947,#207948),(#207949,#207950,#207951),
(#207952,#207953,#207954),(#207955,#207956,#207957)),.UNSPECIFIED.,.F.,
 .F.,.F.)
B_SPLINE_SURFACE_WITH_KNOTS((4,4),(3,3),(0.,0.00039739441082874),(0.,1.),
 .UNSPECIFIED.)
GEOMETRIC_REPRESENTATION_ITEM()
RATIONAL_B_SPLINE_SURFACE(((1.,0.708689770883327,1.),(1.,0.708376440034492,
1.),(1.,0.707750498698403,1.),(1.,0.707106781186548,1.)))
REPRESENTATION_ITEM('')
SURFACE()
);
#3083=(
BOUNDED_SURFACE()
B_SPLINE_SURFACE(3,2,((#207963,#207964,#207965),(#207966,#207967,#207968),
(#207969,#207970,#207971),(#207972,#207973,#207974)),.UNSPECIFIED.,.F.,
 .F.,.F.)
B_SPLINE_SURFACE_WITH_KNOTS((4,4),(3,3),(0.,0.000511815090126179),(0.,1.00105592270391),
 .UNSPECIFIED.)
GEOMETRIC_REPRESENTATION_ITEM()
RATIONAL_B_SPLINE_SURFACE(((1.,0.705266242716965,1.00062243213185),(1.,
0.705584085908659,1.00062176089616),(1.,0.706182089449987,1.00062049800513),
(1.,0.706797508586982,1.00061919833505)))
REPRESENTATION_ITEM('')
SURFACE()
);
#3084=(
BOUNDED_SURFACE()
B_SPLINE_SURFACE(3,2,((#207976,#207977,#207978),(#207979,#207980,#207981),
(#207982,#207983,#207984),(#207985,#207986,#207987)),.UNSPECIFIED.,.F.,
 .F.,.F.)
B_SPLINE_SURFACE_WITH_KNOTS((4,4),(3,3),(0.,0.000397394428086624),(0.,1.),
 .UNSPECIFIED.)
GEOMETRIC_REPRESENTATION_ITEM()
RATIONAL_B_SPLINE_SURFACE(((1.,0.707106781186536,1.),(1.,0.70645984675908,
1.),(1.,0.705820510737281,1.),(1.,0.705498956110757,1.)))
REPRESENTATION_ITEM('')
SURFACE()
);
#3085=(
BOUNDED_SURFACE()
B_SPLINE_SURFACE(3,2,((#207993,#207994,#207995),(#207996,#207997,#207998),
(#207999,#208000,#208001),(#208002,#208003,#208004),(#208005,#208006,#208007),
(#208008,#208009,#208010)),.UNSPECIFIED.,.F.,.F.,.F.)
B_SPLINE_SURFACE_WITH_KNOTS((4,2,4),(3,3),(0.,0.00025795380787285,0.0005159076157457),
(0.,1.),.UNSPECIFIED.)
GEOMETRIC_REPRESENTATION_ITEM()
RATIONAL_B_SPLINE_SURFACE(((1.,0.874619707139398,1.),(1.,0.87483434967915,
1.),(1.,0.854686104157582,1.),(1.,0.79247659791535,1.),(1.,0.750887854594954,
1.),(1.,0.705585838031445,1.)))
REPRESENTATION_ITEM('')
SURFACE()
);
#3086=(
BOUNDED_SURFACE()
B_SPLINE_SURFACE(3,2,((#208016,#208017,#208018),(#208019,#208020,#208021),
(#208022,#208023,#208024),(#208025,#208026,#208027)),.UNSPECIFIED.,.F.,
 .F.,.F.)
B_SPLINE_SURFACE_WITH_KNOTS((4,4),(3,3),(0.,0.000511815437699155),(0.,1.00105881331727),
 .UNSPECIFIED.)
GEOMETRIC_REPRESENTATION_ITEM()
RATIONAL_B_SPLINE_SURFACE(((1.,0.70679666194593,1.000620895198),(1.,0.707430821224804,
1.00061955228542),(1.,0.708058545830307,1.00061822299907),(1.,0.708394505252306,
1.00061751156245)))
REPRESENTATION_ITEM('')
SURFACE()
);
#3087=(
BOUNDED_SURFACE()
B_SPLINE_SURFACE(3,2,((#208029,#208030,#208031),(#208032,#208033,#208034),
(#208035,#208036,#208037),(#208038,#208039,#208040),(#208041,#208042,#208043),
(#208044,#208045,#208046)),.UNSPECIFIED.,.F.,.F.,.F.)
B_SPLINE_SURFACE_WITH_KNOTS((4,2,4),(3,3),(2.71050543121376E-20,0.000256915317531261,
0.000513830635062521),(0.,1.),.UNSPECIFIED.)
GEOMETRIC_REPRESENTATION_ITEM()
RATIONAL_B_SPLINE_SURFACE(((1.,0.705585838031435,1.),(1.,0.75090243354202,
1.),(1.,0.79232953008349,1.),(1.,0.854288401593237,1.),(1.,0.874998031125857,
1.),(1.,0.874619707139389,1.)))
REPRESENTATION_ITEM('')
SURFACE()
);
#3088=(
BOUNDED_SURFACE()
B_SPLINE_SURFACE(3,2,((#208052,#208053,#208054),(#208055,#208056,#208057),
(#208058,#208059,#208060),(#208061,#208062,#208063),(#208064,#208065,#208066),
(#208067,#208068,#208069)),.UNSPECIFIED.,.F.,.F.,.F.)
B_SPLINE_SURFACE_WITH_KNOTS((4,2,4),(3,3),(0.,0.000256592814262156,0.000513185628524312),
(0.,1.),.UNSPECIFIED.)
GEOMETRIC_REPRESENTATION_ITEM()
RATIONAL_B_SPLINE_SURFACE(((1.,0.708712527163647,1.),(1.,0.753780902613735,
1.),(1.,0.79453899576901,1.),(1.,0.855070770331286,1.),(1.,0.875018427445172,
1.),(1.,0.874619707139393,1.)))
REPRESENTATION_ITEM('')
SURFACE()
);
#3089=(
BOUNDED_SURFACE()
B_SPLINE_SURFACE(3,2,((#208071,#208072,#208073),(#208074,#208075,#208076),
(#208077,#208078,#208079),(#208080,#208081,#208082)),.UNSPECIFIED.,.F.,
 .F.,.F.)
B_SPLINE_SURFACE_WITH_KNOTS((4,4),(3,3),(2.71050543121376E-20,0.000511815072430397),
(0.,1.00105598365892),.UNSPECIFIED.)
GEOMETRIC_REPRESENTATION_ITEM()
RATIONAL_B_SPLINE_SURFACE(((1.,0.706797490733671,1.00061923411708),(1.,
0.706182062146594,1.00062053388214),(1.,0.70558406276894,1.00062179683728),
(1.,0.70526622477043,1.00062246810075)))
REPRESENTATION_ITEM('')
SURFACE()
);
#3090=(
BOUNDED_SURFACE()
B_SPLINE_SURFACE(3,2,((#208088,#208089,#208090),(#208091,#208092,#208093),
(#208094,#208095,#208096),(#208097,#208098,#208099),(#208100,#208101,#208102),
(#208103,#208104,#208105)),.UNSPECIFIED.,.F.,.F.,.F.)
B_SPLINE_SURFACE_WITH_KNOTS((4,2,4),(3,3),(-3.34747420754899E-18,0.000257652232350879,
0.000515304464701761),(0.,1.),.UNSPECIFIED.)
GEOMETRIC_REPRESENTATION_ITEM()
RATIONAL_B_SPLINE_SURFACE(((1.,0.874619707139389,1.),(1.,0.874861180430669,
1.),(1.,0.855455725920945,1.),(1.,0.794699358955162,1.),(1.,0.753768977788734,
1.),(1.,0.708712527163667,1.)))
REPRESENTATION_ITEM('')
SURFACE()
);
#3091=(
BOUNDED_SURFACE()
B_SPLINE_SURFACE(3,2,((#208111,#208112,#208113),(#208114,#208115,#208116),
(#208117,#208118,#208119),(#208120,#208121,#208122)),.UNSPECIFIED.,.F.,
 .F.,.F.)
B_SPLINE_SURFACE_WITH_KNOTS((4,4),(3,3),(0.,0.000397394373651905),(0.,1.),
 .UNSPECIFIED.)
GEOMETRIC_REPRESENTATION_ITEM()
RATIONAL_B_SPLINE_SURFACE(((1.,0.707106781186542,1.),(1.,0.707752587915914,
1.),(1.,0.708377654540659,1.),(1.,0.708689770883356,1.)))
REPRESENTATION_ITEM('')
SURFACE()
);
#3092=(
BOUNDED_SURFACE()
B_SPLINE_SURFACE(3,2,((#208124,#208125,#208126),(#208127,#208128,#208129),
(#208130,#208131,#208132),(#208133,#208134,#208135)),.UNSPECIFIED.,.F.,
 .F.,.F.)
B_SPLINE_SURFACE_WITH_KNOTS((4,4),(3,3),(-6.39679281766448E-18,0.000511815456479782),
(0.,1.00105873159862),.UNSPECIFIED.)
GEOMETRIC_REPRESENTATION_ITEM()
RATIONAL_B_SPLINE_SURFACE(((1.,0.708394529056725,1.00061746385284),(1.,
0.708058564167238,1.00061817524612),(1.,0.707430835372476,1.00061950443875),
(1.,0.706796685880768,1.00062084722696)))
REPRESENTATION_ITEM('')
SURFACE()
);
#3093=(
BOUNDED_SURFACE()
B_SPLINE_SURFACE(3,2,((#208141,#208142,#208143),(#208144,#208145,#208146),
(#208147,#208148,#208149),(#208150,#208151,#208152)),.UNSPECIFIED.,.F.,
 .F.,.F.)
B_SPLINE_SURFACE_WITH_KNOTS((4,4),(3,3),(0.,0.000397394465448303),(0.,1.),
 .UNSPECIFIED.)
GEOMETRIC_REPRESENTATION_ITEM()
RATIONAL_B_SPLINE_SURFACE(((1.,0.705498956110748,1.),(1.,0.705821764811772,
1.),(1.,0.706461952521139,1.),(1.,0.707106781186553,1.)))
REPRESENTATION_ITEM('')
SURFACE()
);
#3094=(
BOUNDED_SURFACE()
B_SPLINE_SURFACE(3,2,((#208158,#208159,#208160),(#208161,#208162,#208163),
(#208164,#208165,#208166),(#208167,#208168,#208169)),.UNSPECIFIED.,.F.,
 .F.,.F.)
B_SPLINE_SURFACE_WITH_KNOTS((4,4),(3,3),(0.,0.000397394410828747),(0.,1.),
 .UNSPECIFIED.)
GEOMETRIC_REPRESENTATION_ITEM()
RATIONAL_B_SPLINE_SURFACE(((1.,0.70868977088334,1.),(1.,0.708376440034488,
1.),(1.,0.707750498698412,1.),(1.,0.707106781186555,1.)))
REPRESENTATION_ITEM('')
SURFACE()
);
#3095=(
BOUNDED_SURFACE()
B_SPLINE_SURFACE(3,2,((#208175,#208176,#208177),(#208178,#208179,#208180),
(#208181,#208182,#208183),(#208184,#208185,#208186)),.UNSPECIFIED.,.F.,
 .F.,.F.)
B_SPLINE_SURFACE_WITH_KNOTS((4,4),(3,3),(0.,0.000511815090126184),(0.,1.00105592270487),
 .UNSPECIFIED.)
GEOMETRIC_REPRESENTATION_ITEM()
RATIONAL_B_SPLINE_SURFACE(((1.,0.705266242716691,1.00062243213241),(1.,
0.705584085908343,1.00062176089673),(1.,0.706182089449713,1.00062049800569),
(1.,0.7067975085867,1.00061919833561)))
REPRESENTATION_ITEM('')
SURFACE()
);
#3096=(
BOUNDED_SURFACE()
B_SPLINE_SURFACE(3,2,((#208188,#208189,#208190),(#208191,#208192,#208193),
(#208194,#208195,#208196),(#208197,#208198,#208199)),.UNSPECIFIED.,.F.,
 .F.,.F.)
B_SPLINE_SURFACE_WITH_KNOTS((4,4),(3,3),(0.,0.000397394428086623),(0.,1.),
 .UNSPECIFIED.)
GEOMETRIC_REPRESENTATION_ITEM()
RATIONAL_B_SPLINE_SURFACE(((1.,0.707106781186548,1.),(1.,0.706459846759087,
1.),(1.,0.705820510737271,1.),(1.,0.705498956110752,1.)))
REPRESENTATION_ITEM('')
SURFACE()
);
#3097=(
BOUNDED_SURFACE()
B_SPLINE_SURFACE(3,2,((#208205,#208206,#208207),(#208208,#208209,#208210),
(#208211,#208212,#208213),(#208214,#208215,#208216),(#208217,#208218,#208219),
(#208220,#208221,#208222)),.UNSPECIFIED.,.F.,.F.,.F.)
B_SPLINE_SURFACE_WITH_KNOTS((4,2,4),(3,3),(0.,0.000257953807872843,0.000515907615745687),
(0.,1.),.UNSPECIFIED.)
GEOMETRIC_REPRESENTATION_ITEM()
RATIONAL_B_SPLINE_SURFACE(((1.,0.874619707139384,1.),(1.,0.874834349678893,
1.),(1.,0.854686104157912,1.),(1.,0.792476597915048,1.),(1.,0.750887854595206,
1.),(1.,0.705585838031446,1.)))
REPRESENTATION_ITEM('')
SURFACE()
);
#3098=(
BOUNDED_SURFACE()
B_SPLINE_SURFACE(3,2,((#208228,#208229,#208230),(#208231,#208232,#208233),
(#208234,#208235,#208236),(#208237,#208238,#208239)),.UNSPECIFIED.,.F.,
 .F.,.F.)
B_SPLINE_SURFACE_WITH_KNOTS((4,4),(3,3),(0.,0.000511815437699158),(0.,1.00105881331566),
 .UNSPECIFIED.)
GEOMETRIC_REPRESENTATION_ITEM()
RATIONAL_B_SPLINE_SURFACE(((1.,0.706796661946385,1.00062089519705),(1.,
0.70743082122529,1.00061955228448),(1.,0.708058545830781,1.00061822299813),
(1.,0.708394505252787,1.00061751156151)))
REPRESENTATION_ITEM('')
SURFACE()
);
#3099=(
BOUNDED_SURFACE()
B_SPLINE_SURFACE(3,2,((#208241,#208242,#208243),(#208244,#208245,#208246),
(#208247,#208248,#208249),(#208250,#208251,#208252),(#208253,#208254,#208255),
(#208256,#208257,#208258)),.UNSPECIFIED.,.F.,.F.,.F.)
B_SPLINE_SURFACE_WITH_KNOTS((4,2,4),(3,3),(2.71050543121376E-20,0.00025691531753126,
0.00051383063506252),(0.,1.),.UNSPECIFIED.)
GEOMETRIC_REPRESENTATION_ITEM()
RATIONAL_B_SPLINE_SURFACE(((1.,0.705585838031438,1.),(1.,0.750902433542334,
1.),(1.,0.792329530083076,1.),(1.,0.854288401593664,1.),(1.,0.874998031125545,
1.),(1.,0.874619707139391,1.)))
REPRESENTATION_ITEM('')
SURFACE()
);
#3100=(
BOUNDED_SURFACE()
B_SPLINE_SURFACE(3,2,((#208264,#208265,#208266),(#208267,#208268,#208269),
(#208270,#208271,#208272),(#208273,#208274,#208275),(#208276,#208277,#208278),
(#208279,#208280,#208281)),.UNSPECIFIED.,.F.,.F.,.F.)
B_SPLINE_SURFACE_WITH_KNOTS((4,2,4),(3,3),(0.,0.000256592814262153,0.000513185628524306),
(0.,1.),.UNSPECIFIED.)
GEOMETRIC_REPRESENTATION_ITEM()
RATIONAL_B_SPLINE_SURFACE(((1.,0.708712527163662,1.),(1.,0.753780902613821,
1.),(1.,0.794538995768888,1.),(1.,0.85507077033143,1.),(1.,0.875018427445082,
1.),(1.,0.874619707139386,1.)))
REPRESENTATION_ITEM('')
SURFACE()
);
#3101=(
BOUNDED_SURFACE()
B_SPLINE_SURFACE(3,2,((#208283,#208284,#208285),(#208286,#208287,#208288),
(#208289,#208290,#208291),(#208292,#208293,#208294)),.UNSPECIFIED.,.F.,
 .F.,.F.)
B_SPLINE_SURFACE_WITH_KNOTS((4,4),(3,3),(0.,0.000511815072430401),(0.,1.0010559836604),
 .UNSPECIFIED.)
GEOMETRIC_REPRESENTATION_ITEM()
RATIONAL_B_SPLINE_SURFACE(((1.,0.706797490733232,1.00061923411795),(1.,
0.706182062146145,1.00062053388301),(1.,0.705584062768516,1.00062179683815),
(1.,0.705266224769999,1.00062246810162)))
REPRESENTATION_ITEM('')
SURFACE()
);
#3102=(
BOUNDED_SURFACE()
B_SPLINE_SURFACE(3,2,((#208300,#208301,#208302),(#208303,#208304,#208305),
(#208306,#208307,#208308),(#208309,#208310,#208311),(#208312,#208313,#208314),
(#208315,#208316,#208317)),.UNSPECIFIED.,.F.,.F.,.F.)
B_SPLINE_SURFACE_WITH_KNOTS((4,2,4),(3,3),(0.,0.000257652232350877,0.000515304464701754),
(0.,1.),.UNSPECIFIED.)
GEOMETRIC_REPRESENTATION_ITEM()
RATIONAL_B_SPLINE_SURFACE(((1.,0.874619707139387,1.),(1.,0.874861180430517,
1.),(1.,0.855455725921104,1.),(1.,0.794699358955021,1.),(1.,0.753768977788863,
1.),(1.,0.708712527163641,1.)))
REPRESENTATION_ITEM('')
SURFACE()
);
#3103=(
BOUNDED_SURFACE()
B_SPLINE_SURFACE(3,2,((#208323,#208324,#208325),(#208326,#208327,#208328),
(#208329,#208330,#208331),(#208332,#208333,#208334)),.UNSPECIFIED.,.F.,
 .F.,.F.)
B_SPLINE_SURFACE_WITH_KNOTS((4,4),(3,3),(0.,0.000397394373651908),(0.,1.),
 .UNSPECIFIED.)
GEOMETRIC_REPRESENTATION_ITEM()
RATIONAL_B_SPLINE_SURFACE(((1.,0.707106781186556,1.),(1.,0.707752587915904,
1.),(1.,0.708377654540669,1.),(1.,0.708689770883336,1.)))
REPRESENTATION_ITEM('')
SURFACE()
);
#3104=(
BOUNDED_SURFACE()
B_SPLINE_SURFACE(3,2,((#208336,#208337,#208338),(#208339,#208340,#208341),
(#208342,#208343,#208344),(#208345,#208346,#208347)),.UNSPECIFIED.,.F.,
 .F.,.F.)
B_SPLINE_SURFACE_WITH_KNOTS((4,4),(3,3),(0.,0.000511815456479792),(0.,1.00105873160375),
 .UNSPECIFIED.)
GEOMETRIC_REPRESENTATION_ITEM()
RATIONAL_B_SPLINE_SURFACE(((1.,0.708394529055219,1.00061746385583),(1.,
0.708058564165767,1.00061817524912),(1.,0.707430835370929,1.00061950444175),
(1.,0.706796685879273,1.00062084722997)))
REPRESENTATION_ITEM('')
SURFACE()
);
#3105=(
BOUNDED_SURFACE()
B_SPLINE_SURFACE(3,2,((#208353,#208354,#208355),(#208356,#208357,#208358),
(#208359,#208360,#208361),(#208362,#208363,#208364)),.UNSPECIFIED.,.F.,
 .F.,.F.)
B_SPLINE_SURFACE_WITH_KNOTS((4,4),(3,3),(0.,0.0003973944654483),(0.,1.),
 .UNSPECIFIED.)
GEOMETRIC_REPRESENTATION_ITEM()
RATIONAL_B_SPLINE_SURFACE(((1.,0.70549895611075,1.),(1.,0.705821764811787,
1.),(1.,0.70646195252115,1.),(1.,0.707106781186548,1.)))
REPRESENTATION_ITEM('')
SURFACE()
);
#3106=(
BOUNDED_SURFACE()
B_SPLINE_SURFACE(3,2,((#208370,#208371,#208372),(#208373,#208374,#208375),
(#208376,#208377,#208378),(#208379,#208380,#208381)),.UNSPECIFIED.,.F.,
 .F.,.F.)
B_SPLINE_SURFACE_WITH_KNOTS((4,4),(3,3),(0.,0.000397394410828731),(0.,1.),
 .UNSPECIFIED.)
GEOMETRIC_REPRESENTATION_ITEM()
RATIONAL_B_SPLINE_SURFACE(((1.,0.708689770883321,1.),(1.,0.708376440034497,
1.),(1.,0.707750498698426,1.),(1.,0.707106781186538,1.)))
REPRESENTATION_ITEM('')
SURFACE()
);
#3107=(
BOUNDED_SURFACE()
B_SPLINE_SURFACE(3,2,((#208387,#208388,#208389),(#208390,#208391,#208392),
(#208393,#208394,#208395),(#208396,#208397,#208398)),.UNSPECIFIED.,.F.,
 .F.,.F.)
B_SPLINE_SURFACE_WITH_KNOTS((4,4),(3,3),(0.,0.000511815090126176),(0.,1.0010559227031),
 .UNSPECIFIED.)
GEOMETRIC_REPRESENTATION_ITEM()
RATIONAL_B_SPLINE_SURFACE(((1.,0.705266242717241,1.00062243213137),(1.,
0.705584085908851,1.00062176089569),(1.,0.70618208945024,1.00062049800466),
(1.,0.706797508587208,1.00061919833458)))
REPRESENTATION_ITEM('')
SURFACE()
);
#3108=(
BOUNDED_SURFACE()
B_SPLINE_SURFACE(3,2,((#208400,#208401,#208402),(#208403,#208404,#208405),
(#208406,#208407,#208408),(#208409,#208410,#208411)),.UNSPECIFIED.,.F.,
 .F.,.F.)
B_SPLINE_SURFACE_WITH_KNOTS((4,4),(3,3),(-1.52872506320456E-17,0.000397394428086609),
(0.,1.),.UNSPECIFIED.)
GEOMETRIC_REPRESENTATION_ITEM()
RATIONAL_B_SPLINE_SURFACE(((1.,0.707106781186549,1.),(1.,0.706459846759096,
1.),(1.,0.705820510737299,1.),(1.,0.705498956110724,1.)))
REPRESENTATION_ITEM('')
SURFACE()
);
#3109=(
BOUNDED_SURFACE()
B_SPLINE_SURFACE(3,2,((#208417,#208418,#208419),(#208420,#208421,#208422),
(#208423,#208424,#208425),(#208426,#208427,#208428),(#208429,#208430,#208431),
(#208432,#208433,#208434)),.UNSPECIFIED.,.F.,.F.,.F.)
B_SPLINE_SURFACE_WITH_KNOTS((4,2,4),(3,3),(0.,0.000257953807872847,0.000515907615745694),
(0.,1.),.UNSPECIFIED.)
GEOMETRIC_REPRESENTATION_ITEM()
RATIONAL_B_SPLINE_SURFACE(((1.,0.874619707139391,1.),(1.,0.874834349679487,
1.),(1.,0.854686104157114,1.),(1.,0.792476597915844,1.),(1.,0.75088785459459,
1.),(1.,0.705585838031461,1.)))
REPRESENTATION_ITEM('')
SURFACE()
);
#3110=(
BOUNDED_SURFACE()
B_SPLINE_SURFACE(3,2,((#208440,#208441,#208442),(#208443,#208444,#208445),
(#208446,#208447,#208448),(#208449,#208450,#208451)),.UNSPECIFIED.,.F.,
 .F.,.F.)
B_SPLINE_SURFACE_WITH_KNOTS((4,4),(3,3),(0.,0.000511815437699146),(0.,1.00105881331828),
 .UNSPECIFIED.)
GEOMETRIC_REPRESENTATION_ITEM()
RATIONAL_B_SPLINE_SURFACE(((1.,0.706796661945634,1.00062089519859),(1.,
0.707430821224513,1.00061955228601),(1.,0.708058545830029,1.00061822299966),
(1.,0.708394505252009,1.00061751156304)))
REPRESENTATION_ITEM('')
SURFACE()
);
#3111=(
BOUNDED_SURFACE()
B_SPLINE_SURFACE(3,2,((#208453,#208454,#208455),(#208456,#208457,#208458),
(#208459,#208460,#208461),(#208462,#208463,#208464),(#208465,#208466,#208467),
(#208468,#208469,#208470)),.UNSPECIFIED.,.F.,.F.,.F.)
B_SPLINE_SURFACE_WITH_KNOTS((4,2,4),(3,3),(0.,0.000256915317531259,0.000513830635062518),
(0.,1.),.UNSPECIFIED.)
GEOMETRIC_REPRESENTATION_ITEM()
RATIONAL_B_SPLINE_SURFACE(((1.,0.705585838031464,1.),(1.,0.750902433542663,
1.),(1.,0.792329530082664,1.),(1.,0.854288401594055,1.),(1.,0.874998031125273,
1.),(1.,0.874619707139395,1.)))
REPRESENTATION_ITEM('')
SURFACE()
);
#3112=(
BOUNDED_SURFACE()
B_SPLINE_SURFACE(3,2,((#208476,#208477,#208478),(#208479,#208480,#208481),
(#208482,#208483,#208484),(#208485,#208486,#208487),(#208488,#208489,#208490),
(#208491,#208492,#208493)),.UNSPECIFIED.,.F.,.F.,.F.)
B_SPLINE_SURFACE_WITH_KNOTS((4,2,4),(3,3),(0.,0.000256592814262156,0.000513185628524312),
(0.,1.),.UNSPECIFIED.)
GEOMETRIC_REPRESENTATION_ITEM()
RATIONAL_B_SPLINE_SURFACE(((1.,0.708712527163668,1.),(1.,0.753780902613508,
1.),(1.,0.794538995769307,1.),(1.,0.855070770330991,1.),(1.,0.875018427445403,
1.),(1.,0.874619707139386,1.)))
REPRESENTATION_ITEM('')
SURFACE()
);
#3113=(
BOUNDED_SURFACE()
B_SPLINE_SURFACE(3,2,((#208495,#208496,#208497),(#208498,#208499,#208500),
(#208501,#208502,#208503),(#208504,#208505,#208506)),.UNSPECIFIED.,.F.,
 .F.,.F.)
B_SPLINE_SURFACE_WITH_KNOTS((4,4),(3,3),(0.,0.000511815072430389),(0.,1.00105598366069),
 .UNSPECIFIED.)
GEOMETRIC_REPRESENTATION_ITEM()
RATIONAL_B_SPLINE_SURFACE(((1.,0.706797490733162,1.00061923411812),(1.,
0.706182062146082,1.00062053388318),(1.,0.705584062768414,1.00062179683833),
(1.,0.705266224769911,1.00062246810179)))
REPRESENTATION_ITEM('')
SURFACE()
);
#3114=(
BOUNDED_SURFACE()
B_SPLINE_SURFACE(3,2,((#208512,#208513,#208514),(#208515,#208516,#208517),
(#208518,#208519,#208520),(#208521,#208522,#208523),(#208524,#208525,#208526),
(#208527,#208528,#208529)),.UNSPECIFIED.,.F.,.F.,.F.)
B_SPLINE_SURFACE_WITH_KNOTS((4,2,4),(3,3),(0.,0.000257652232350886,0.000515304464701772),
(0.,1.),.UNSPECIFIED.)
GEOMETRIC_REPRESENTATION_ITEM()
RATIONAL_B_SPLINE_SURFACE(((1.,0.874619707139379,1.),(1.,0.874861180430367,
1.),(1.,0.855455725921303,1.),(1.,0.794699358954818,1.),(1.,0.753768977788941,
1.),(1.,0.708712527163667,1.)))
REPRESENTATION_ITEM('')
SURFACE()
);
#3115=(
BOUNDED_SURFACE()
B_SPLINE_SURFACE(3,2,((#208535,#208536,#208537),(#208538,#208539,#208540),
(#208541,#208542,#208543),(#208544,#208545,#208546)),.UNSPECIFIED.,.F.,
 .F.,.F.)
B_SPLINE_SURFACE_WITH_KNOTS((4,4),(3,3),(-1.53143556863578E-17,0.000397394373651904),
(0.,1.),.UNSPECIFIED.)
GEOMETRIC_REPRESENTATION_ITEM()
RATIONAL_B_SPLINE_SURFACE(((1.,0.707106781186548,1.),(1.,0.707752587915843,
1.),(1.,0.70837765454073,1.),(1.,0.708689770883302,1.)))
REPRESENTATION_ITEM('')
SURFACE()
);
#3116=(
BOUNDED_SURFACE()
B_SPLINE_SURFACE(3,2,((#208548,#208549,#208550),(#208551,#208552,#208553),
(#208554,#208555,#208556),(#208557,#208558,#208559)),.UNSPECIFIED.,.F.,
 .F.,.F.)
B_SPLINE_SURFACE_WITH_KNOTS((4,4),(3,3),(0.,0.000511815456479788),(0.,1.0010587315999),
 .UNSPECIFIED.)
GEOMETRIC_REPRESENTATION_ITEM()
RATIONAL_B_SPLINE_SURFACE(((1.,0.708394529056346,1.00061746385358),(1.,
0.70805856416687,1.00061817524687),(1.,0.707430835372085,1.00061950443949),
(1.,0.706796685880394,1.00062084722771)))
REPRESENTATION_ITEM('')
SURFACE()
);
#3117=(
BOUNDED_SURFACE()
B_SPLINE_SURFACE(3,2,((#208565,#208566,#208567),(#208568,#208569,#208570),
(#208571,#208572,#208573),(#208574,#208575,#208576)),.UNSPECIFIED.,.F.,
 .F.,.F.)
B_SPLINE_SURFACE_WITH_KNOTS((4,4),(3,3),(0.,0.000397394465448305),(0.,1.),
 .UNSPECIFIED.)
GEOMETRIC_REPRESENTATION_ITEM()
RATIONAL_B_SPLINE_SURFACE(((1.,0.705498956110757,1.),(1.,0.705821764811778,
1.),(1.,0.70646195252114,1.),(1.,0.707106781186556,1.)))
REPRESENTATION_ITEM('')
SURFACE()
);
#3118=(
BOUNDED_SURFACE()
B_SPLINE_SURFACE(3,2,((#208582,#208583,#208584),(#208585,#208586,#208587),
(#208588,#208589,#208590),(#208591,#208592,#208593)),.UNSPECIFIED.,.F.,
 .F.,.F.)
B_SPLINE_SURFACE_WITH_KNOTS((4,4),(3,3),(0.,0.000397394410828738),(0.,1.),
 .UNSPECIFIED.)
GEOMETRIC_REPRESENTATION_ITEM()
RATIONAL_B_SPLINE_SURFACE(((1.,0.708689770883337,1.),(1.,0.708376440034459,
1.),(1.,0.707750498698444,1.),(1.,0.707106781186536,1.)))
REPRESENTATION_ITEM('')
SURFACE()
);
#3119=(
BOUNDED_SURFACE()
B_SPLINE_SURFACE(3,2,((#208599,#208600,#208601),(#208602,#208603,#208604),
(#208605,#208606,#208607),(#208608,#208609,#208610)),.UNSPECIFIED.,.F.,
 .F.,.F.)
B_SPLINE_SURFACE_WITH_KNOTS((4,4),(3,3),(0.,0.000511815090126175),(0.,1.00105592270252),
 .UNSPECIFIED.)
GEOMETRIC_REPRESENTATION_ITEM()
RATIONAL_B_SPLINE_SURFACE(((1.,0.705266242717401,1.00062243213103),(1.,
0.705584085909057,1.00062176089535),(1.,0.70618208945039,1.00062049800432),
(1.,0.706797508587387,1.00061919833424)))
REPRESENTATION_ITEM('')
SURFACE()
);
#3120=(
BOUNDED_SURFACE()
B_SPLINE_SURFACE(3,2,((#208612,#208613,#208614),(#208615,#208616,#208617),
(#208618,#208619,#208620),(#208621,#208622,#208623)),.UNSPECIFIED.,.F.,
 .F.,.F.)
B_SPLINE_SURFACE_WITH_KNOTS((4,4),(3,3),(0.,0.000397394428086644),(0.,1.),
 .UNSPECIFIED.)
GEOMETRIC_REPRESENTATION_ITEM()
RATIONAL_B_SPLINE_SURFACE(((1.,0.707106781186536,1.),(1.,0.706459846759106,
1.),(1.,0.705820510737281,1.),(1.,0.705498956110761,1.)))
REPRESENTATION_ITEM('')
SURFACE()
);
#3121=(
BOUNDED_SURFACE()
B_SPLINE_SURFACE(3,2,((#208629,#208630,#208631),(#208632,#208633,#208634),
(#208635,#208636,#208637),(#208638,#208639,#208640),(#208641,#208642,#208643),
(#208644,#208645,#208646)),.UNSPECIFIED.,.F.,.F.,.F.)
B_SPLINE_SURFACE_WITH_KNOTS((4,2,4),(3,3),(0.,0.000257953807872846,0.000515907615745692),
(0.,1.),.UNSPECIFIED.)
GEOMETRIC_REPRESENTATION_ITEM()
RATIONAL_B_SPLINE_SURFACE(((1.,0.87461970713939,1.),(1.,0.874834349679058,
1.),(1.,0.854686104157715,1.),(1.,0.792476597915225,1.),(1.,0.750887854595065,
1.),(1.,0.705585838031458,1.)))
REPRESENTATION_ITEM('')
SURFACE()
);
#3122=(
BOUNDED_SURFACE()
B_SPLINE_SURFACE(3,2,((#208652,#208653,#208654),(#208655,#208656,#208657),
(#208658,#208659,#208660),(#208661,#208662,#208663)),.UNSPECIFIED.,.F.,
 .F.,.F.)
B_SPLINE_SURFACE_WITH_KNOTS((4,4),(3,3),(0.,0.000511815437699154),(0.,1.00105881331964),
 .UNSPECIFIED.)
GEOMETRIC_REPRESENTATION_ITEM()
RATIONAL_B_SPLINE_SURFACE(((1.,0.706796661945235,1.00062089519939),(1.,
0.707430821224115,1.00061955228681),(1.,0.708058545829616,1.00061822300046),
(1.,0.708394505251623,1.00061751156384)))
REPRESENTATION_ITEM('')
SURFACE()
);
#3123=(
BOUNDED_SURFACE()
B_SPLINE_SURFACE(3,2,((#208665,#208666,#208667),(#208668,#208669,#208670),
(#208671,#208672,#208673),(#208674,#208675,#208676),(#208677,#208678,#208679),
(#208680,#208681,#208682)),.UNSPECIFIED.,.F.,.F.,.F.)
B_SPLINE_SURFACE_WITH_KNOTS((4,2,4),(3,3),(0.,0.000256915317531264,0.000513830635062528),
(0.,1.),.UNSPECIFIED.)
GEOMETRIC_REPRESENTATION_ITEM()
RATIONAL_B_SPLINE_SURFACE(((1.,0.705585838031448,1.),(1.,0.75090243354285,
1.),(1.,0.792329530082401,1.),(1.,0.854288401594319,1.),(1.,0.874998031125059,
1.),(1.,0.874619707139403,1.)))
REPRESENTATION_ITEM('')
SURFACE()
);
#3124=(
BOUNDED_SURFACE()
B_SPLINE_SURFACE(3,2,((#208688,#208689,#208690),(#208691,#208692,#208693),
(#208694,#208695,#208696),(#208697,#208698,#208699),(#208700,#208701,#208702),
(#208703,#208704,#208705)),.UNSPECIFIED.,.F.,.F.,.F.)
B_SPLINE_SURFACE_WITH_KNOTS((4,2,4),(3,3),(-9.45966395493603E-18,0.000256592814262146,
0.000513185628524302),(0.,1.),.UNSPECIFIED.)
GEOMETRIC_REPRESENTATION_ITEM()
RATIONAL_B_SPLINE_SURFACE(((1.,0.708712527163665,1.),(1.,0.753780902613326,
1.),(1.,0.794538995769537,1.),(1.,0.855070770330762,1.),(1.,0.875018427445575,
1.),(1.,0.874619707139397,1.)))
REPRESENTATION_ITEM('')
SURFACE()
);
#3125=(
BOUNDED_SURFACE()
B_SPLINE_SURFACE(3,2,((#208707,#208708,#208709),(#208710,#208711,#208712),
(#208713,#208714,#208715),(#208716,#208717,#208718)),.UNSPECIFIED.,.F.,
 .F.,.F.)
B_SPLINE_SURFACE_WITH_KNOTS((4,4),(3,3),(0.,0.000511815072430404),(0.,1.00105598365946),
 .UNSPECIFIED.)
GEOMETRIC_REPRESENTATION_ITEM()
RATIONAL_B_SPLINE_SURFACE(((1.,0.706797490733526,1.0006192341174),(1.,0.706182062146386,
1.00062053388246),(1.,0.705584062768819,1.0006217968376),(1.,0.705266224770269,
1.00062246810107)))
REPRESENTATION_ITEM('')
SURFACE()
);
#3126=(
BOUNDED_SURFACE()
B_SPLINE_SURFACE(3,2,((#208724,#208725,#208726),(#208727,#208728,#208729),
(#208730,#208731,#208732),(#208733,#208734,#208735),(#208736,#208737,#208738),
(#208739,#208740,#208741)),.UNSPECIFIED.,.F.,.F.,.F.)
B_SPLINE_SURFACE_WITH_KNOTS((4,2,4),(3,3),(0.,0.000257652232350881,0.000515304464701762),
(0.,1.),.UNSPECIFIED.)
GEOMETRIC_REPRESENTATION_ITEM()
RATIONAL_B_SPLINE_SURFACE(((1.,0.874619707139382,1.),(1.,0.874861180430684,
1.),(1.,0.855455725920868,1.),(1.,0.794699358955249,1.),(1.,0.753768977788646,
1.),(1.,0.708712527163657,1.)))
REPRESENTATION_ITEM('')
SURFACE()
);
#3127=(
BOUNDED_SURFACE()
B_SPLINE_SURFACE(3,2,((#208747,#208748,#208749),(#208750,#208751,#208752),
(#208753,#208754,#208755),(#208756,#208757,#208758)),.UNSPECIFIED.,.F.,
 .F.,.F.)
B_SPLINE_SURFACE_WITH_KNOTS((4,4),(3,3),(0.,0.000397394373651921),(0.,1.),
 .UNSPECIFIED.)
GEOMETRIC_REPRESENTATION_ITEM()
RATIONAL_B_SPLINE_SURFACE(((1.,0.707106781186548,1.),(1.,0.707752587915883,
1.),(1.,0.708377654540729,1.),(1.,0.708689770883306,1.)))
REPRESENTATION_ITEM('')
SURFACE()
);
#3128=(
BOUNDED_SURFACE()
B_SPLINE_SURFACE(3,2,((#208760,#208761,#208762),(#208763,#208764,#208765),
(#208766,#208767,#208768),(#208769,#208770,#208771)),.UNSPECIFIED.,.F.,
 .F.,.F.)
B_SPLINE_SURFACE_WITH_KNOTS((4,4),(3,3),(-6.42389787197661E-18,0.000511815456479787),
(0.,1.00105873159917),.UNSPECIFIED.)
GEOMETRIC_REPRESENTATION_ITEM()
RATIONAL_B_SPLINE_SURFACE(((1.,0.708394529056561,1.00061746385316),(1.,
0.708058564167106,1.00061817524645),(1.,0.707430835372293,1.00061950443907),
(1.,0.706796685880606,1.00062084722728)))
REPRESENTATION_ITEM('')
SURFACE()
);
#3129=(
BOUNDED_SURFACE()
B_SPLINE_SURFACE(3,2,((#208777,#208778,#208779),(#208780,#208781,#208782),
(#208783,#208784,#208785),(#208786,#208787,#208788)),.UNSPECIFIED.,.F.,
 .F.,.F.)
B_SPLINE_SURFACE_WITH_KNOTS((4,4),(3,3),(0.,0.000397394465448318),(0.,1.),
 .UNSPECIFIED.)
GEOMETRIC_REPRESENTATION_ITEM()
RATIONAL_B_SPLINE_SURFACE(((1.,0.705498956110736,1.),(1.,0.705821764811785,
1.),(1.,0.706461952521153,1.),(1.,0.707106781186548,1.)))
REPRESENTATION_ITEM('')
SURFACE()
);
#3130=(
BOUNDED_SURFACE()
B_SPLINE_SURFACE(3,2,((#208794,#208795,#208796),(#208797,#208798,#208799),
(#208800,#208801,#208802),(#208803,#208804,#208805)),.UNSPECIFIED.,.F.,
 .F.,.F.)
B_SPLINE_SURFACE_WITH_KNOTS((4,4),(3,3),(0.,0.000397394410828749),(0.,1.),
 .UNSPECIFIED.)
GEOMETRIC_REPRESENTATION_ITEM()
RATIONAL_B_SPLINE_SURFACE(((1.,0.708689770883341,1.),(1.,0.708376440034476,
1.),(1.,0.707750498698437,1.),(1.,0.707106781186548,1.)))
REPRESENTATION_ITEM('')
SURFACE()
);
#3131=(
BOUNDED_SURFACE()
B_SPLINE_SURFACE(3,2,((#208811,#208812,#208813),(#208814,#208815,#208816),
(#208817,#208818,#208819),(#208820,#208821,#208822)),.UNSPECIFIED.,.F.,
 .F.,.F.)
B_SPLINE_SURFACE_WITH_KNOTS((4,4),(3,3),(-6.42389787197661E-18,0.000511815090126168),
(0.,1.00105592270135),.UNSPECIFIED.)
GEOMETRIC_REPRESENTATION_ITEM()
RATIONAL_B_SPLINE_SURFACE(((1.,0.705266242717731,1.00062243213034),(1.,
0.705584085909352,1.00062176089466),(1.,0.706182089450749,1.00062049800363),
(1.,0.70679750858773,1.00061919833355)))
REPRESENTATION_ITEM('')
SURFACE()
);
#3132=(
BOUNDED_SURFACE()
B_SPLINE_SURFACE(3,2,((#208824,#208825,#208826),(#208827,#208828,#208829),
(#208830,#208831,#208832),(#208833,#208834,#208835)),.UNSPECIFIED.,.F.,
 .F.,.F.)
B_SPLINE_SURFACE_WITH_KNOTS((4,4),(3,3),(-9.64939933512099E-18,0.00039739442808662),
(0.,1.),.UNSPECIFIED.)
GEOMETRIC_REPRESENTATION_ITEM()
RATIONAL_B_SPLINE_SURFACE(((1.,0.707106781186548,1.),(1.,0.70645984675908,
1.),(1.,0.705820510737268,1.),(1.,0.705498956110742,1.)))
REPRESENTATION_ITEM('')
SURFACE()
);
#3133=(
BOUNDED_SURFACE()
B_SPLINE_SURFACE(3,2,((#208841,#208842,#208843),(#208844,#208845,#208846),
(#208847,#208848,#208849),(#208850,#208851,#208852),(#208853,#208854,#208855),
(#208856,#208857,#208858)),.UNSPECIFIED.,.F.,.F.,.F.)
B_SPLINE_SURFACE_WITH_KNOTS((4,2,4),(3,3),(0.,0.00025795380787284,0.00051590761574568),
(0.,1.),.UNSPECIFIED.)
GEOMETRIC_REPRESENTATION_ITEM()
RATIONAL_B_SPLINE_SURFACE(((1.,0.874619707139388,1.),(1.,0.874834349678587,
1.),(1.,0.854686104158307,1.),(1.,0.792476597914645,1.),(1.,0.750887854595489,
1.),(1.,0.705585838031426,1.)))
REPRESENTATION_ITEM('')
SURFACE()
);
#3134=(
BOUNDED_SURFACE()
B_SPLINE_SURFACE(3,2,((#208864,#208865,#208866),(#208867,#208868,#208869),
(#208870,#208871,#208872),(#208873,#208874,#208875)),.UNSPECIFIED.,.F.,
 .F.,.F.)
B_SPLINE_SURFACE_WITH_KNOTS((4,4),(3,3),(0.,0.000511815437699152),(0.,1.00105881331964),
 .UNSPECIFIED.)
GEOMETRIC_REPRESENTATION_ITEM()
RATIONAL_B_SPLINE_SURFACE(((1.,0.706796661945223,1.00062089519939),(1.,
0.707430821224125,1.00061955228681),(1.,0.708058545829633,1.00061822300046),
(1.,0.708394505251633,1.00061751156384)))
REPRESENTATION_ITEM('')
SURFACE()
);
#3135=(
BOUNDED_SURFACE()
B_SPLINE_SURFACE(3,2,((#208877,#208878,#208879),(#208880,#208881,#208882),
(#208883,#208884,#208885),(#208886,#208887,#208888),(#208889,#208890,#208891),
(#208892,#208893,#208894)),.UNSPECIFIED.,.F.,.F.,.F.)
B_SPLINE_SURFACE_WITH_KNOTS((4,2,4),(3,3),(0.,0.000256915317531262,0.000513830635062523),
(0.,1.),.UNSPECIFIED.)
GEOMETRIC_REPRESENTATION_ITEM()
RATIONAL_B_SPLINE_SURFACE(((1.,0.705585838031437,1.),(1.,0.750902433543188,
1.),(1.,0.792329530081924,1.),(1.,0.854288401594778,1.),(1.,0.874998031124709,
1.),(1.,0.87461970713939,1.)))
REPRESENTATION_ITEM('')
SURFACE()
);
#3136=(
BOUNDED_SURFACE()
B_SPLINE_SURFACE(3,2,((#208900,#208901,#208902),(#208903,#208904,#208905),
(#208906,#208907,#208908),(#208909,#208910,#208911),(#208912,#208913,#208914),
(#208915,#208916,#208917)),.UNSPECIFIED.,.F.,.F.,.F.)
B_SPLINE_SURFACE_WITH_KNOTS((4,2,4),(3,3),(-9.32413868337534E-18,0.00025659281426215,
0.000513185628524309),(0.,1.),.UNSPECIFIED.)
GEOMETRIC_REPRESENTATION_ITEM()
RATIONAL_B_SPLINE_SURFACE(((1.,0.708712527163675,1.),(1.,0.753780902613439,
1.),(1.,0.794538995769399,1.),(1.,0.855070770330883,1.),(1.,0.875018427445492,
1.),(1.,0.874619707139387,1.)))
REPRESENTATION_ITEM('')
SURFACE()
);
#3137=(
BOUNDED_SURFACE()
B_SPLINE_SURFACE(3,2,((#208919,#208920,#208921),(#208922,#208923,#208924),
(#208925,#208926,#208927),(#208928,#208929,#208930)),.UNSPECIFIED.,.F.,
 .F.,.F.)
B_SPLINE_SURFACE_WITH_KNOTS((4,4),(3,3),(-5.09575021068187E-18,0.000511815072430393),
(0.,1.0010559836582),.UNSPECIFIED.)
GEOMETRIC_REPRESENTATION_ITEM()
RATIONAL_B_SPLINE_SURFACE(((1.,0.706797490733882,1.00061923411666),(1.,
0.7061820621468,1.00062053388172),(1.,0.705584062769178,1.00062179683686),
(1.,0.705266224770652,1.00062246810032)))
REPRESENTATION_ITEM('')
SURFACE()
);
#3138=(
BOUNDED_SURFACE()
B_SPLINE_SURFACE(3,2,((#208936,#208937,#208938),(#208939,#208940,#208941),
(#208942,#208943,#208944),(#208945,#208946,#208947),(#208948,#208949,#208950),
(#208951,#208952,#208953)),.UNSPECIFIED.,.F.,.F.,.F.)
B_SPLINE_SURFACE_WITH_KNOTS((4,2,4),(3,3),(0.,0.000257652232350884,0.000515304464701767),
(0.,1.),.UNSPECIFIED.)
GEOMETRIC_REPRESENTATION_ITEM()
RATIONAL_B_SPLINE_SURFACE(((1.,0.874619707139388,1.),(1.,0.87486118043046,
1.),(1.,0.855455725921212,1.),(1.,0.7946993589549,1.),(1.,0.753768977788974,
1.),(1.,0.708712527163625,1.)))
REPRESENTATION_ITEM('')
SURFACE()
);
#3139=(
BOUNDED_SURFACE()
B_SPLINE_SURFACE(3,2,((#208959,#208960,#208961),(#208962,#208963,#208964),
(#208965,#208966,#208967),(#208968,#208969,#208970)),.UNSPECIFIED.,.F.,
 .F.,.F.)
B_SPLINE_SURFACE_WITH_KNOTS((4,4),(3,3),(-1.47451495458029E-17,0.000397394373651904),
(0.,1.),.UNSPECIFIED.)
GEOMETRIC_REPRESENTATION_ITEM()
RATIONAL_B_SPLINE_SURFACE(((1.,0.70710678118656,1.),(1.,0.707752587915888,
1.),(1.,0.708377654540624,1.),(1.,0.708689770883349,1.)))
REPRESENTATION_ITEM('')
SURFACE()
);
#3140=(
BOUNDED_SURFACE()
B_SPLINE_SURFACE(3,2,((#208972,#208973,#208974),(#208975,#208976,#208977),
(#208978,#208979,#208980),(#208981,#208982,#208983)),.UNSPECIFIED.,.F.,
 .F.,.F.)
B_SPLINE_SURFACE_WITH_KNOTS((4,4),(3,3),(0.,0.000511815456479796),(0.,1.00105873159821),
 .UNSPECIFIED.)
GEOMETRIC_REPRESENTATION_ITEM()
RATIONAL_B_SPLINE_SURFACE(((1.,0.708394529056829,1.0006174638526),(1.,0.708058564167371,
1.00061817524589),(1.,0.707430835372575,1.00061950443851),(1.,0.706796685880887,
1.00062084722672)))
REPRESENTATION_ITEM('')
SURFACE()
);
#3141=(
BOUNDED_SURFACE()
B_SPLINE_SURFACE(3,2,((#208989,#208990,#208991),(#208992,#208993,#208994),
(#208995,#208996,#208997),(#208998,#208999,#209000)),.UNSPECIFIED.,.F.,
 .F.,.F.)
B_SPLINE_SURFACE_WITH_KNOTS((4,4),(3,3),(-6.50521303491303E-18,0.000397394465448302),
(0.,1.),.UNSPECIFIED.)
GEOMETRIC_REPRESENTATION_ITEM()
RATIONAL_B_SPLINE_SURFACE(((1.,0.705498956110765,1.),(1.,0.70582176481176,
1.),(1.,0.706461952521179,1.),(1.,0.707106781186535,1.)))
REPRESENTATION_ITEM('')
SURFACE()
);
#3142=(
BOUNDED_SURFACE()
B_SPLINE_SURFACE(3,2,((#209006,#209007,#209008),(#209009,#209010,#209011),
(#209012,#209013,#209014),(#209015,#209016,#209017)),.UNSPECIFIED.,.F.,
 .F.,.F.)
B_SPLINE_SURFACE_WITH_KNOTS((4,4),(3,3),(0.,0.000397394410828735),(0.,1.),
 .UNSPECIFIED.)
GEOMETRIC_REPRESENTATION_ITEM()
RATIONAL_B_SPLINE_SURFACE(((1.,0.708689770883313,1.),(1.,0.708376440034517,
1.),(1.,0.707750498698387,1.),(1.,0.707106781186548,1.)))
REPRESENTATION_ITEM('')
SURFACE()
);
#3143=(
BOUNDED_SURFACE()
B_SPLINE_SURFACE(3,2,((#209023,#209024,#209025),(#209026,#209027,#209028),
(#209029,#209030,#209031),(#209032,#209033,#209034)),.UNSPECIFIED.,.F.,
 .F.,.F.)
B_SPLINE_SURFACE_WITH_KNOTS((4,4),(3,3),(0.,0.000511815090126171),(0.,1.00105592270182),
 .UNSPECIFIED.)
GEOMETRIC_REPRESENTATION_ITEM()
RATIONAL_B_SPLINE_SURFACE(((1.,0.705266242717594,1.00062243213061),(1.,
0.705584085909257,1.00062176089493),(1.,0.706182089450605,1.0006204980039),
(1.,0.706797508587594,1.00061919833382)))
REPRESENTATION_ITEM('')
SURFACE()
);
#3144=(
BOUNDED_SURFACE()
B_SPLINE_SURFACE(3,2,((#209036,#209037,#209038),(#209039,#209040,#209041),
(#209042,#209043,#209044),(#209045,#209046,#209047)),.UNSPECIFIED.,.F.,
 .F.,.F.)
B_SPLINE_SURFACE_WITH_KNOTS((4,4),(3,3),(-9.64939933512099E-18,0.000397394428086625),
(0.,1.),.UNSPECIFIED.)
GEOMETRIC_REPRESENTATION_ITEM()
RATIONAL_B_SPLINE_SURFACE(((1.,0.707106781186548,1.),(1.,0.706459846759098,
1.),(1.,0.705820510737279,1.),(1.,0.705498956110752,1.)))
REPRESENTATION_ITEM('')
SURFACE()
);
#3145=(
BOUNDED_SURFACE()
B_SPLINE_SURFACE(3,2,((#209053,#209054,#209055),(#209056,#209057,#209058),
(#209059,#209060,#209061),(#209062,#209063,#209064),(#209065,#209066,#209067),
(#209068,#209069,#209070)),.UNSPECIFIED.,.F.,.F.,.F.)
B_SPLINE_SURFACE_WITH_KNOTS((4,2,4),(3,3),(0.,0.000257953807872847,0.000515907615745693),
(0.,1.),.UNSPECIFIED.)
GEOMETRIC_REPRESENTATION_ITEM()
RATIONAL_B_SPLINE_SURFACE(((1.,0.874619707139394,1.),(1.,0.87483434967884,
1.),(1.,0.85468610415798,1.),(1.,0.792476597914961,1.),(1.,0.75088785459526,
1.),(1.,0.705585838031473,1.)))
REPRESENTATION_ITEM('')
SURFACE()
);
#3146=(
BOUNDED_SURFACE()
B_SPLINE_SURFACE(3,2,((#209076,#209077,#209078),(#209079,#209080,#209081),
(#209082,#209083,#209084),(#209085,#209086,#209087)),.UNSPECIFIED.,.F.,
 .F.,.F.)
B_SPLINE_SURFACE_WITH_KNOTS((4,4),(3,3),(0.,0.000511815437699157),(0.,1.00105881331725),
 .UNSPECIFIED.)
GEOMETRIC_REPRESENTATION_ITEM()
RATIONAL_B_SPLINE_SURFACE(((1.,0.706796661945923,1.00062089519799),(1.,
0.707430821224819,1.00061955228541),(1.,0.708058545830314,1.00061822299906),
(1.,0.708394505252314,1.00061751156244)))
REPRESENTATION_ITEM('')
SURFACE()
);
#3147=(
BOUNDED_SURFACE()
B_SPLINE_SURFACE(3,2,((#209089,#209090,#209091),(#209092,#209093,#209094),
(#209095,#209096,#209097),(#209098,#209099,#209100),(#209101,#209102,#209103),
(#209104,#209105,#209106)),.UNSPECIFIED.,.F.,.F.,.F.)
B_SPLINE_SURFACE_WITH_KNOTS((4,2,4),(3,3),(2.71050543121376E-20,0.000256915317531264,
0.000513830635062527),(0.,1.),.UNSPECIFIED.)
GEOMETRIC_REPRESENTATION_ITEM()
RATIONAL_B_SPLINE_SURFACE(((1.,0.705585838031416,1.),(1.,0.750902433542516,
1.),(1.,0.792329530082844,1.),(1.,0.854288401593844,1.),(1.,0.874998031125403,
1.),(1.,0.874619707139391,1.)))
REPRESENTATION_ITEM('')
SURFACE()
);
#3148=(
BOUNDED_SURFACE()
B_SPLINE_SURFACE(3,2,((#209112,#209113,#209114),(#209115,#209116,#209117),
(#209118,#209119,#209120),(#209121,#209122,#209123),(#209124,#209125,#209126),
(#209127,#209128,#209129)),.UNSPECIFIED.,.F.,.F.,.F.)
B_SPLINE_SURFACE_WITH_KNOTS((4,2,4),(3,3),(0.,0.000256592814262161,0.000513185628524323),
(0.,1.),.UNSPECIFIED.)
GEOMETRIC_REPRESENTATION_ITEM()
RATIONAL_B_SPLINE_SURFACE(((1.,0.70871252716366,1.),(1.,0.753780902613878,
1.),(1.,0.794538995768779,1.),(1.,0.855070770331533,1.),(1.,0.875018427445003,
1.),(1.,0.874619707139393,1.)))
REPRESENTATION_ITEM('')
SURFACE()
);
#3149=(
BOUNDED_SURFACE()
B_SPLINE_SURFACE(3,2,((#209131,#209132,#209133),(#209134,#209135,#209136),
(#209137,#209138,#209139),(#209140,#209141,#209142)),.UNSPECIFIED.,.F.,
 .F.,.F.)
B_SPLINE_SURFACE_WITH_KNOTS((4,4),(3,3),(-5.06864515636973E-18,0.000511815072430401),
(0.,1.00105598365977),.UNSPECIFIED.)
GEOMETRIC_REPRESENTATION_ITEM()
RATIONAL_B_SPLINE_SURFACE(((1.,0.706797490733424,1.00061923411758),(1.,
0.706182062146334,1.00062053388264),(1.,0.705584062768699,1.00062179683778),
(1.,0.705266224770158,1.00062246810125)))
REPRESENTATION_ITEM('')
SURFACE()
);
#3150=(
BOUNDED_SURFACE()
B_SPLINE_SURFACE(3,2,((#209148,#209149,#209150),(#209151,#209152,#209153),
(#209154,#209155,#209156),(#209157,#209158,#209159),(#209160,#209161,#209162),
(#209163,#209164,#209165)),.UNSPECIFIED.,.F.,.F.,.F.)
B_SPLINE_SURFACE_WITH_KNOTS((4,2,4),(3,3),(1.35525271560688E-20,0.000257652232350885,
0.00051530446470177),(0.,1.),.UNSPECIFIED.)
GEOMETRIC_REPRESENTATION_ITEM()
RATIONAL_B_SPLINE_SURFACE(((1.,0.874619707139391,1.),(1.,0.874861180430548,
1.),(1.,0.855455725921059,1.),(1.,0.79469935895508,1.),(1.,0.753768977788768,
1.),(1.,0.708712527163675,1.)))
REPRESENTATION_ITEM('')
SURFACE()
);
#3151=(
BOUNDED_SURFACE()
B_SPLINE_SURFACE(3,2,((#209171,#209172,#209173),(#209174,#209175,#209176),
(#209177,#209178,#209179),(#209180,#209181,#209182)),.UNSPECIFIED.,.F.,
 .F.,.F.)
B_SPLINE_SURFACE_WITH_KNOTS((4,4),(3,3),(0.,0.000397394373651914),(0.,1.),
 .UNSPECIFIED.)
GEOMETRIC_REPRESENTATION_ITEM()
RATIONAL_B_SPLINE_SURFACE(((1.,0.707106781186535,1.),(1.,0.707752587915914,
1.),(1.,0.708377654540683,1.),(1.,0.708689770883326,1.)))
REPRESENTATION_ITEM('')
SURFACE()
);
#3152=(
BOUNDED_SURFACE()
B_SPLINE_SURFACE(3,2,((#209184,#209185,#209186),(#209187,#209188,#209189),
(#209190,#209191,#209192),(#209193,#209194,#209195)),.UNSPECIFIED.,.F.,
 .F.,.F.)
B_SPLINE_SURFACE_WITH_KNOTS((4,4),(3,3),(0.,0.000511815456479784),(0.,1.00105873159912),
 .UNSPECIFIED.)
GEOMETRIC_REPRESENTATION_ITEM()
RATIONAL_B_SPLINE_SURFACE(((1.,0.708394529056566,1.00061746385313),(1.,
0.708058564167135,1.00061817524642),(1.,0.707430835372306,1.00061950443904),
(1.,0.706796685880622,1.00062084722725)))
REPRESENTATION_ITEM('')
SURFACE()
);
#3153=(
BOUNDED_SURFACE()
B_SPLINE_SURFACE(3,2,((#209201,#209202,#209203),(#209204,#209205,#209206),
(#209207,#209208,#209209),(#209210,#209211,#209212)),.UNSPECIFIED.,.F.,
 .F.,.F.)
B_SPLINE_SURFACE_WITH_KNOTS((4,4),(3,3),(0.,0.000397394465448309),(0.,1.),
 .UNSPECIFIED.)
GEOMETRIC_REPRESENTATION_ITEM()
RATIONAL_B_SPLINE_SURFACE(((1.,0.705498956110767,1.),(1.,0.705821764811776,
1.),(1.,0.706461952521138,1.),(1.,0.707106781186548,1.)))
REPRESENTATION_ITEM('')
SURFACE()
);
#3154=(
BOUNDED_SURFACE()
B_SPLINE_SURFACE(3,2,((#209218,#209219,#209220),(#209221,#209222,#209223),
(#209224,#209225,#209226),(#209227,#209228,#209229)),.UNSPECIFIED.,.F.,
 .F.,.F.)
B_SPLINE_SURFACE_WITH_KNOTS((4,4),(3,3),(0.,0.000397394410828743),(0.,1.),
 .UNSPECIFIED.)
GEOMETRIC_REPRESENTATION_ITEM()
RATIONAL_B_SPLINE_SURFACE(((1.,0.708689770883332,1.),(1.,0.708376440034505,
1.),(1.,0.707750498698407,1.),(1.,0.707106781186548,1.)))
REPRESENTATION_ITEM('')
SURFACE()
);
#3155=(
BOUNDED_SURFACE()
B_SPLINE_SURFACE(3,2,((#209235,#209236,#209237),(#209238,#209239,#209240),
(#209241,#209242,#209243),(#209244,#209245,#209246)),.UNSPECIFIED.,.F.,
 .F.,.F.)
B_SPLINE_SURFACE_WITH_KNOTS((4,4),(3,3),(0.,0.000511815090126178),(0.,1.00105592270222),
 .UNSPECIFIED.)
GEOMETRIC_REPRESENTATION_ITEM()
RATIONAL_B_SPLINE_SURFACE(((1.,0.705266242717482,1.00062243213085),(1.,
0.705584085909123,1.00062176089517),(1.,0.706182089450473,1.00062049800414),
(1.,0.706797508587475,1.00061919833406)))
REPRESENTATION_ITEM('')
SURFACE()
);
#3156=(
BOUNDED_SURFACE()
B_SPLINE_SURFACE(3,2,((#209248,#209249,#209250),(#209251,#209252,#209253),
(#209254,#209255,#209256),(#209257,#209258,#209259)),.UNSPECIFIED.,.F.,
 .F.,.F.)
B_SPLINE_SURFACE_WITH_KNOTS((4,4),(3,3),(0.,0.000397394428086621),(0.,1.),
 .UNSPECIFIED.)
GEOMETRIC_REPRESENTATION_ITEM()
RATIONAL_B_SPLINE_SURFACE(((1.,0.707106781186548,1.),(1.,0.706459846759103,
1.),(1.,0.705820510737277,1.),(1.,0.705498956110743,1.)))
REPRESENTATION_ITEM('')
SURFACE()
);
#3157=(
BOUNDED_SURFACE()
B_SPLINE_SURFACE(3,2,((#209265,#209266,#209267),(#209268,#209269,#209270),
(#209271,#209272,#209273),(#209274,#209275,#209276),(#209277,#209278,#209279),
(#209280,#209281,#209282)),.UNSPECIFIED.,.F.,.F.,.F.)
B_SPLINE_SURFACE_WITH_KNOTS((4,2,4),(3,3),(-9.6900569165892E-18,0.00025795380787284,
0.00051590761574569),(0.,1.),.UNSPECIFIED.)
GEOMETRIC_REPRESENTATION_ITEM()
RATIONAL_B_SPLINE_SURFACE(((1.,0.874619707139392,1.),(1.,0.8748343496787,
1.),(1.,0.854686104158173,1.),(1.,0.792476597914769,1.),(1.,0.750887854595394,
1.),(1.,0.705585838031444,1.)))
REPRESENTATION_ITEM('')
SURFACE()
);
#3158=(
BOUNDED_SURFACE()
B_SPLINE_SURFACE(3,2,((#209288,#209289,#209290),(#209291,#209292,#209293),
(#209294,#209295,#209296),(#209297,#209298,#209299)),.UNSPECIFIED.,.F.,
 .F.,.F.)
B_SPLINE_SURFACE_WITH_KNOTS((4,4),(3,3),(0.,0.000511815437699158),(0.,1.00105881331441),
 .UNSPECIFIED.)
GEOMETRIC_REPRESENTATION_ITEM()
RATIONAL_B_SPLINE_SURFACE(((1.,0.706796661946769,1.00062089519632),(1.,
0.707430821225625,1.00061955228374),(1.,0.708058545831196,1.0006182229974),
(1.,0.708394505253119,1.00061751156078)))
REPRESENTATION_ITEM('')
SURFACE()
);
#3159=(
BOUNDED_SURFACE()
B_SPLINE_SURFACE(3,2,((#209301,#209302,#209303),(#209304,#209305,#209306),
(#209307,#209308,#209309),(#209310,#209311,#209312),(#209313,#209314,#209315),
(#209316,#209317,#209318)),.UNSPECIFIED.,.F.,.F.,.F.)
B_SPLINE_SURFACE_WITH_KNOTS((4,2,4),(3,3),(0.,0.000256915317531254,0.000513830635062507),
(0.,1.),.UNSPECIFIED.)
GEOMETRIC_REPRESENTATION_ITEM()
RATIONAL_B_SPLINE_SURFACE(((1.,0.705585838031438,1.),(1.,0.750902433543063,
1.),(1.,0.792329530082044,1.),(1.,0.854288401594628,1.),(1.,0.874998031124815,
1.),(1.,0.874619707139389,1.)))
REPRESENTATION_ITEM('')
SURFACE()
);
#3160=(
BOUNDED_SURFACE()
B_SPLINE_SURFACE(3,2,((#209324,#209325,#209326),(#209327,#209328,#209329),
(#209330,#209331,#209332),(#209333,#209334,#209335),(#209336,#209337,#209338),
(#209339,#209340,#209341)),.UNSPECIFIED.,.F.,.F.,.F.)
B_SPLINE_SURFACE_WITH_KNOTS((4,2,4),(3,3),(-8.94466792300541E-18,0.000256592814262149,
0.000513185628524306),(0.,1.),.UNSPECIFIED.)
GEOMETRIC_REPRESENTATION_ITEM()
RATIONAL_B_SPLINE_SURFACE(((1.,0.708712527163696,1.),(1.,0.753780902613059,
1.),(1.,0.794538995769904,1.),(1.,0.855070770330386,1.),(1.,0.875018427445873,
1.),(1.,0.874619707139387,1.)))
REPRESENTATION_ITEM('')
SURFACE()
);
#3161=(
BOUNDED_SURFACE()
B_SPLINE_SURFACE(3,2,((#209343,#209344,#209345),(#209346,#209347,#209348),
(#209349,#209350,#209351),(#209352,#209353,#209354)),.UNSPECIFIED.,.F.,
 .F.,.F.)
B_SPLINE_SURFACE_WITH_KNOTS((4,4),(3,3),(-5.52943107967607E-18,0.000511815072430393),
(0.,1.0010559836602),.UNSPECIFIED.)
GEOMETRIC_REPRESENTATION_ITEM()
RATIONAL_B_SPLINE_SURFACE(((1.,0.706797490733287,1.00061923411783),(1.,
0.706182062146219,1.00062053388289),(1.,0.705584062768592,1.00062179683803),
(1.,0.705266224770059,1.0006224681015)))
REPRESENTATION_ITEM('')
SURFACE()
);
#3162=(
BOUNDED_SURFACE()
B_SPLINE_SURFACE(3,2,((#209360,#209361,#209362),(#209363,#209364,#209365),
(#209366,#209367,#209368),(#209369,#209370,#209371),(#209372,#209373,#209374),
(#209375,#209376,#209377)),.UNSPECIFIED.,.F.,.F.,.F.)
B_SPLINE_SURFACE_WITH_KNOTS((4,2,4),(3,3),(1.35525271560688E-20,0.000257652232350877,
0.000515304464701754),(0.,1.),.UNSPECIFIED.)
GEOMETRIC_REPRESENTATION_ITEM()
RATIONAL_B_SPLINE_SURFACE(((1.,0.874619707139397,1.),(1.,0.874861180430313,
1.),(1.,0.855455725921391,1.),(1.,0.79469935895477,1.),(1.,0.753768977788991,
1.),(1.,0.708712527163673,1.)))
REPRESENTATION_ITEM('')
SURFACE()
);
#3163=(
BOUNDED_SURFACE()
B_SPLINE_SURFACE(3,2,((#209383,#209384,#209385),(#209386,#209387,#209388),
(#209389,#209390,#209391),(#209392,#209393,#209394)),.UNSPECIFIED.,.F.,
 .F.,.F.)
B_SPLINE_SURFACE_WITH_KNOTS((4,4),(3,3),(0.,0.000397394373651919),(0.,1.),
 .UNSPECIFIED.)
GEOMETRIC_REPRESENTATION_ITEM()
RATIONAL_B_SPLINE_SURFACE(((1.,0.707106781186559,1.),(1.,0.707752587915881,
1.),(1.,0.708377654540695,1.),(1.,0.70868977088332,1.)))
REPRESENTATION_ITEM('')
SURFACE()
);
#3164=(
BOUNDED_SURFACE()
B_SPLINE_SURFACE(3,2,((#209396,#209397,#209398),(#209399,#209400,#209401),
(#209402,#209403,#209404),(#209405,#209406,#209407)),.UNSPECIFIED.,.F.,
 .F.,.F.)
B_SPLINE_SURFACE_WITH_KNOTS((4,4),(3,3),(0.,0.000511815456479789),(0.,1.00105873160043),
 .UNSPECIFIED.)
GEOMETRIC_REPRESENTATION_ITEM()
RATIONAL_B_SPLINE_SURFACE(((1.,0.708394529056183,1.00061746385389),(1.,
0.70805856416675,1.00061817524718),(1.,0.707430835371893,1.00061950443981),
(1.,0.706796685880238,1.00062084722802)))
REPRESENTATION_ITEM('')
SURFACE()
);
#3165=(
BOUNDED_SURFACE()
B_SPLINE_SURFACE(3,2,((#209413,#209414,#209415),(#209416,#209417,#209418),
(#209419,#209420,#209421),(#209422,#209423,#209424)),.UNSPECIFIED.,.F.,
 .F.,.F.)
B_SPLINE_SURFACE_WITH_KNOTS((4,4),(3,3),(-6.50521303491303E-18,0.000397394465448301),
(0.,1.),.UNSPECIFIED.)
GEOMETRIC_REPRESENTATION_ITEM()
RATIONAL_B_SPLINE_SURFACE(((1.,0.705498956110777,1.),(1.,0.705821764811791,
1.),(1.,0.706461952521121,1.),(1.,0.707106781186559,1.)))
REPRESENTATION_ITEM('')
SURFACE()
);
#3166=(
BOUNDED_SURFACE()
B_SPLINE_SURFACE(3,2,((#209430,#209431,#209432),(#209433,#209434,#209435),
(#209436,#209437,#209438),(#209439,#209440,#209441)),.UNSPECIFIED.,.F.,
 .F.,.F.)
B_SPLINE_SURFACE_WITH_KNOTS((4,4),(3,3),(0.,0.000397394410828737),(0.,1.),
 .UNSPECIFIED.)
GEOMETRIC_REPRESENTATION_ITEM()
RATIONAL_B_SPLINE_SURFACE(((1.,0.708689770883354,1.),(1.,0.708376440034479,
1.),(1.,0.707750498698412,1.),(1.,0.707106781186548,1.)))
REPRESENTATION_ITEM('')
SURFACE()
);
#3167=(
BOUNDED_SURFACE()
B_SPLINE_SURFACE(3,2,((#209447,#209448,#209449),(#209450,#209451,#209452),
(#209453,#209454,#209455),(#209456,#209457,#209458)),.UNSPECIFIED.,.F.,
 .F.,.F.)
B_SPLINE_SURFACE_WITH_KNOTS((4,4),(3,3),(0.,0.000511815090126188),(0.,1.0010559227012),
 .UNSPECIFIED.)
GEOMETRIC_REPRESENTATION_ITEM()
RATIONAL_B_SPLINE_SURFACE(((1.,0.705266242717776,1.00062243213025),(1.,
0.705584085909439,1.00062176089456),(1.,0.706182089450786,1.00062049800353),
(1.,0.706797508587776,1.00061919833346)))
REPRESENTATION_ITEM('')
SURFACE()
);
#3168=(
BOUNDED_SURFACE()
B_SPLINE_SURFACE(3,2,((#209460,#209461,#209462),(#209463,#209464,#209465),
(#209466,#209467,#209468),(#209469,#209470,#209471)),.UNSPECIFIED.,.F.,
 .F.,.F.)
B_SPLINE_SURFACE_WITH_KNOTS((4,4),(3,3),(-1.69948690537103E-17,0.000397394428086611),
(0.,1.),.UNSPECIFIED.)
GEOMETRIC_REPRESENTATION_ITEM()
RATIONAL_B_SPLINE_SURFACE(((1.,0.707106781186546,1.),(1.,0.706459846759102,
1.),(1.,0.705820510737254,1.),(1.,0.70549895611076,1.)))
REPRESENTATION_ITEM('')
SURFACE()
);
#3169=(
BOUNDED_SURFACE()
B_SPLINE_SURFACE(3,2,((#209477,#209478,#209479),(#209480,#209481,#209482),
(#209483,#209484,#209485),(#209486,#209487,#209488),(#209489,#209490,#209491),
(#209492,#209493,#209494)),.UNSPECIFIED.,.F.,.F.,.F.)
B_SPLINE_SURFACE_WITH_KNOTS((4,2,4),(3,3),(0.,0.000257953807872847,0.000515907615745694),
(0.,1.),.UNSPECIFIED.)
GEOMETRIC_REPRESENTATION_ITEM()
RATIONAL_B_SPLINE_SURFACE(((1.,0.874619707139392,1.),(1.,0.874834349679603,
1.),(1.,0.854686104156984,1.),(1.,0.792476597915974,1.),(1.,0.750887854594486,
1.),(1.,0.705585838031442,1.)))
REPRESENTATION_ITEM('')
SURFACE()
);
#3170=(
BOUNDED_SURFACE()
B_SPLINE_SURFACE(3,2,((#209500,#209501,#209502),(#209503,#209504,#209505),
(#209506,#209507,#209508),(#209509,#209510,#209511)),.UNSPECIFIED.,.F.,
 .F.,.F.)
B_SPLINE_SURFACE_WITH_KNOTS((4,4),(3,3),(0.,0.000511815437699155),(0.,1.00105881331789),
 .UNSPECIFIED.)
GEOMETRIC_REPRESENTATION_ITEM()
RATIONAL_B_SPLINE_SURFACE(((1.,0.706796661945747,1.00062089519837),(1.,
0.707430821224615,1.00061955228579),(1.,0.708058545830165,1.00061822299944),
(1.,0.708394505252133,1.00061751156282)))
REPRESENTATION_ITEM('')
SURFACE()
);
#3171=(
BOUNDED_SURFACE()
B_SPLINE_SURFACE(3,2,((#209513,#209514,#209515),(#209516,#209517,#209518),
(#209519,#209520,#209521),(#209522,#209523,#209524),(#209525,#209526,#209527),
(#209528,#209529,#209530)),.UNSPECIFIED.,.F.,.F.,.F.)
B_SPLINE_SURFACE_WITH_KNOTS((4,2,4),(3,3),(0.,0.000256915317531267,0.000513830635062534),
(0.,1.),.UNSPECIFIED.)
GEOMETRIC_REPRESENTATION_ITEM()
RATIONAL_B_SPLINE_SURFACE(((1.,0.705585838031445,1.),(1.,0.75090243354203,
1.),(1.,0.792329530083494,1.),(1.,0.854288401593243,1.),(1.,0.874998031125855,
1.),(1.,0.874619707139413,1.)))
REPRESENTATION_ITEM('')
SURFACE()
);
#3172=(
BOUNDED_SURFACE()
B_SPLINE_SURFACE(3,2,((#209536,#209537,#209538),(#209539,#209540,#209541),
(#209542,#209543,#209544),(#209545,#209546,#209547),(#209548,#209549,#209550),
(#209551,#209552,#209553)),.UNSPECIFIED.,.F.,.F.,.F.)
B_SPLINE_SURFACE_WITH_KNOTS((4,2,4),(3,3),(-7.23704950134074E-18,0.000256592814262153,
0.000513185628524314),(0.,1.),.UNSPECIFIED.)
GEOMETRIC_REPRESENTATION_ITEM()
RATIONAL_B_SPLINE_SURFACE(((1.,0.708712527163663,1.),(1.,0.753780902613181,
1.),(1.,0.794538995769752,1.),(1.,0.855070770330559,1.),(1.,0.875018427445738,
1.),(1.,0.874619707139388,1.)))
REPRESENTATION_ITEM('')
SURFACE()
);
#3173=(
BOUNDED_SURFACE()
B_SPLINE_SURFACE(3,2,((#209555,#209556,#209557),(#209558,#209559,#209560),
(#209561,#209562,#209563),(#209564,#209565,#209566)),.UNSPECIFIED.,.F.,
 .F.,.F.)
B_SPLINE_SURFACE_WITH_KNOTS((4,4),(3,3),(0.,0.000511815072430406),(0.,1.001055983659),
 .UNSPECIFIED.)
GEOMETRIC_REPRESENTATION_ITEM()
RATIONAL_B_SPLINE_SURFACE(((1.,0.706797490733647,1.00061923411713),(1.,
0.706182062146584,1.00062053388219),(1.,0.705584062768908,1.00062179683733),
(1.,0.70526622477043,1.0006224681008)))
REPRESENTATION_ITEM('')
SURFACE()
);
#3174=(
BOUNDED_SURFACE()
B_SPLINE_SURFACE(3,2,((#209572,#209573,#209574),(#209575,#209576,#209577),
(#209578,#209579,#209580),(#209581,#209582,#209583),(#209584,#209585,#209586),
(#209587,#209588,#209589)),.UNSPECIFIED.,.F.,.F.,.F.)
B_SPLINE_SURFACE_WITH_KNOTS((4,2,4),(3,3),(0.,0.000257652232350887,0.000515304464701775),
(0.,1.),.UNSPECIFIED.)
GEOMETRIC_REPRESENTATION_ITEM()
RATIONAL_B_SPLINE_SURFACE(((1.,0.874619707139375,1.),(1.,0.874861180430142,
1.),(1.,0.8554557259216,1.),(1.,0.7946993589545,1.),(1.,0.753768977789186,
1.),(1.,0.708712527163656,1.)))
REPRESENTATION_ITEM('')
SURFACE()
);
#3175=(
BOUNDED_SURFACE()
B_SPLINE_SURFACE(3,2,((#209595,#209596,#209597),(#209598,#209599,#209600),
(#209601,#209602,#209603),(#209604,#209605,#209606)),.UNSPECIFIED.,.F.,
 .F.,.F.)
B_SPLINE_SURFACE_WITH_KNOTS((4,4),(3,3),(0.,0.000397394373651914),(0.,1.),
 .UNSPECIFIED.)
GEOMETRIC_REPRESENTATION_ITEM()
RATIONAL_B_SPLINE_SURFACE(((1.,0.707106781186558,1.),(1.,0.707752587915874,
1.),(1.,0.708377654540684,1.),(1.,0.708689770883325,1.)))
REPRESENTATION_ITEM('')
SURFACE()
);
#3176=(
BOUNDED_SURFACE()
B_SPLINE_SURFACE(3,2,((#209608,#209609,#209610),(#209611,#209612,#209613),
(#209614,#209615,#209616),(#209617,#209618,#209619)),.UNSPECIFIED.,.F.,
 .F.,.F.)
B_SPLINE_SURFACE_WITH_KNOTS((4,4),(3,3),(0.,0.000511815456479791),(0.,1.00105873160094),
 .UNSPECIFIED.)
GEOMETRIC_REPRESENTATION_ITEM()
RATIONAL_B_SPLINE_SURFACE(((1.,0.708394529056042,1.00061746385419),(1.,
0.7080585641666,1.00061817524748),(1.,0.707430835371753,1.0006195044401),
(1.,0.706796685880089,1.00062084722832)))
REPRESENTATION_ITEM('')
SURFACE()
);
#3177=(
BOUNDED_SURFACE()
B_SPLINE_SURFACE(3,2,((#209625,#209626,#209627),(#209628,#209629,#209630),
(#209631,#209632,#209633),(#209634,#209635,#209636)),.UNSPECIFIED.,.F.,
 .F.,.F.)
B_SPLINE_SURFACE_WITH_KNOTS((4,4),(3,3),(0.,0.00039739446544832),(0.,1.),
 .UNSPECIFIED.)
GEOMETRIC_REPRESENTATION_ITEM()
RATIONAL_B_SPLINE_SURFACE(((1.,0.705498956110787,1.),(1.,0.705821764811737,
1.),(1.,0.706461952521161,1.),(1.,0.707106781186548,1.)))
REPRESENTATION_ITEM('')
SURFACE()
);
#3178=(
BOUNDED_SURFACE()
B_SPLINE_SURFACE(3,2,((#209642,#209643,#209644),(#209645,#209646,#209647),
(#209648,#209649,#209650),(#209651,#209652,#209653)),.UNSPECIFIED.,.F.,
 .F.,.F.)
B_SPLINE_SURFACE_WITH_KNOTS((4,4),(3,3),(0.,0.000397394410828738),(0.,1.),
 .UNSPECIFIED.)
GEOMETRIC_REPRESENTATION_ITEM()
RATIONAL_B_SPLINE_SURFACE(((1.,0.708689770883308,1.),(1.,0.708376440034552,
1.),(1.,0.707750498698383,1.),(1.,0.707106781186548,1.)))
REPRESENTATION_ITEM('')
SURFACE()
);
#3179=(
BOUNDED_SURFACE()
B_SPLINE_SURFACE(3,2,((#209659,#209660,#209661),(#209662,#209663,#209664),
(#209665,#209666,#209667),(#209668,#209669,#209670)),.UNSPECIFIED.,.F.,
 .F.,.F.)
B_SPLINE_SURFACE_WITH_KNOTS((4,4),(3,3),(0.,0.000511815090126185),(0.,1.00105592270171),
 .UNSPECIFIED.)
GEOMETRIC_REPRESENTATION_ITEM()
RATIONAL_B_SPLINE_SURFACE(((1.,0.705266242717622,1.00062243213055),(1.,
0.705584085909267,1.00062176089486),(1.,0.706182089450651,1.00062049800383),
(1.,0.706797508587617,1.00061919833376)))
REPRESENTATION_ITEM('')
SURFACE()
);
#3180=(
BOUNDED_SURFACE()
B_SPLINE_SURFACE(3,2,((#209672,#209673,#209674),(#209675,#209676,#209677),
(#209678,#209679,#209680),(#209681,#209682,#209683)),.UNSPECIFIED.,.F.,
 .F.,.F.)
B_SPLINE_SURFACE_WITH_KNOTS((4,4),(3,3),(-7.61652026171067E-18,0.000397394428086623),
(0.,1.),.UNSPECIFIED.)
GEOMETRIC_REPRESENTATION_ITEM()
RATIONAL_B_SPLINE_SURFACE(((1.,0.707106781186548,1.),(1.,0.7064598467591,
1.),(1.,0.705820510737261,1.),(1.,0.705498956110754,1.)))
REPRESENTATION_ITEM('')
SURFACE()
);
#3181=(
BOUNDED_SURFACE()
B_SPLINE_SURFACE(3,2,((#209689,#209690,#209691),(#209692,#209693,#209694),
(#209695,#209696,#209697),(#209698,#209699,#209700),(#209701,#209702,#209703),
(#209704,#209705,#209706)),.UNSPECIFIED.,.F.,.F.,.F.)
B_SPLINE_SURFACE_WITH_KNOTS((4,2,4),(3,3),(0.,0.000257953807872849,0.000515907615745698),
(0.,1.),.UNSPECIFIED.)
GEOMETRIC_REPRESENTATION_ITEM()
RATIONAL_B_SPLINE_SURFACE(((1.,0.874619707139392,1.),(1.,0.8748343496791,
1.),(1.,0.854686104157651,1.),(1.,0.792476597915266,1.),(1.,0.750887854595039,
1.),(1.,0.705585838031425,1.)))
REPRESENTATION_ITEM('')
SURFACE()
);
#3182=(
BOUNDED_SURFACE()
B_SPLINE_SURFACE(3,2,((#209712,#209713,#209714),(#209715,#209716,#209717),
(#209718,#209719,#209720),(#209721,#209722,#209723)),.UNSPECIFIED.,.F.,
 .F.,.F.)
B_SPLINE_SURFACE_WITH_KNOTS((4,4),(3,3),(0.,0.000511815437699155),(0.,1.00105881331537),
 .UNSPECIFIED.)
GEOMETRIC_REPRESENTATION_ITEM()
RATIONAL_B_SPLINE_SURFACE(((1.,0.706796661946478,1.00062089519688),(1.,
0.707430821225356,1.00061955228431),(1.,0.708058545830873,1.00061822299797),
(1.,0.708394505252873,1.00061751156135)))
REPRESENTATION_ITEM('')
SURFACE()
);
#3183=(
BOUNDED_SURFACE()
B_SPLINE_SURFACE(3,2,((#209725,#209726,#209727),(#209728,#209729,#209730),
(#209731,#209732,#209733),(#209734,#209735,#209736),(#209737,#209738,#209739),
(#209740,#209741,#209742)),.UNSPECIFIED.,.F.,.F.,.F.)
B_SPLINE_SURFACE_WITH_KNOTS((4,2,4),(3,3),(0.,0.000256915317531255,0.00051383063506251),
(0.,1.),.UNSPECIFIED.)
GEOMETRIC_REPRESENTATION_ITEM()
RATIONAL_B_SPLINE_SURFACE(((1.,0.705585838031433,1.),(1.,0.750902433542673,
1.),(1.,0.792329530082634,1.),(1.,0.854288401594081,1.),(1.,0.874998031125218,
1.),(1.,0.874619707139388,1.)))
REPRESENTATION_ITEM('')
SURFACE()
);
#3184=(
BOUNDED_SURFACE()
B_SPLINE_SURFACE(3,2,((#209748,#209749,#209750),(#209751,#209752,#209753),
(#209754,#209755,#209756),(#209757,#209758,#209759),(#209760,#209761,#209762),
(#209763,#209764,#209765)),.UNSPECIFIED.,.F.,.F.,.F.)
B_SPLINE_SURFACE_WITH_KNOTS((4,2,4),(3,3),(-7.10152422978005E-18,0.000256592814262155,
0.000513185628524318),(0.,1.),.UNSPECIFIED.)
GEOMETRIC_REPRESENTATION_ITEM()
RATIONAL_B_SPLINE_SURFACE(((1.,0.708712527163678,1.),(1.,0.753780902613814,
1.),(1.,0.794538995768887,1.),(1.,0.855070770331403,1.),(1.,0.875018427445105,
1.),(1.,0.874619707139391,1.)))
REPRESENTATION_ITEM('')
SURFACE()
);
#3185=(
BOUNDED_SURFACE()
B_SPLINE_SURFACE(3,2,((#209767,#209768,#209769),(#209770,#209771,#209772),
(#209773,#209774,#209775),(#209776,#209777,#209778)),.UNSPECIFIED.,.F.,
 .F.,.F.)
B_SPLINE_SURFACE_WITH_KNOTS((4,4),(3,3),(0.,0.000511815072430409),(0.,1.00105598366036),
 .UNSPECIFIED.)
GEOMETRIC_REPRESENTATION_ITEM()
RATIONAL_B_SPLINE_SURFACE(((1.,0.706797490733251,1.00061923411792),(1.,
0.706182062146167,1.00062053388299),(1.,0.705584062768538,1.00062179683813),
(1.,0.70526622477001,1.0006224681016)))
REPRESENTATION_ITEM('')
SURFACE()
);
#3186=(
BOUNDED_SURFACE()
B_SPLINE_SURFACE(3,2,((#209784,#209785,#209786),(#209787,#209788,#209789),
(#209790,#209791,#209792),(#209793,#209794,#209795),(#209796,#209797,#209798),
(#209799,#209800,#209801)),.UNSPECIFIED.,.F.,.F.,.F.)
B_SPLINE_SURFACE_WITH_KNOTS((4,2,4),(3,3),(-2.99510850149121E-18,0.000257652232350881,
0.000515304464701765),(0.,1.),.UNSPECIFIED.)
GEOMETRIC_REPRESENTATION_ITEM()
RATIONAL_B_SPLINE_SURFACE(((1.,0.87461970713939,1.),(1.,0.874861180430529,
1.),(1.,0.855455725921095,1.),(1.,0.794699358955062,1.),(1.,0.75376897778881,
1.),(1.,0.708712527163653,1.)))
REPRESENTATION_ITEM('')
SURFACE()
);
#3187=(
BOUNDED_SURFACE()
B_SPLINE_SURFACE(3,2,((#209807,#209808,#209809),(#209810,#209811,#209812),
(#209813,#209814,#209815),(#209816,#209817,#209818)),.UNSPECIFIED.,.F.,
 .F.,.F.)
B_SPLINE_SURFACE_WITH_KNOTS((4,4),(3,3),(0.,0.000397394373651926),(0.,1.),
 .UNSPECIFIED.)
GEOMETRIC_REPRESENTATION_ITEM()
RATIONAL_B_SPLINE_SURFACE(((1.,0.707106781186548,1.),(1.,0.70775258791589,
1.),(1.,0.708377654540707,1.),(1.,0.708689770883312,1.)))
REPRESENTATION_ITEM('')
SURFACE()
);
#3188=(
BOUNDED_SURFACE()
B_SPLINE_SURFACE(3,2,((#209820,#209821,#209822),(#209823,#209824,#209825),
(#209826,#209827,#209828),(#209829,#209830,#209831)),.UNSPECIFIED.,.F.,
 .F.,.F.)
B_SPLINE_SURFACE_WITH_KNOTS((4,4),(3,3),(0.,0.000511815456479792),(0.,1.00105873159908),
 .UNSPECIFIED.)
GEOMETRIC_REPRESENTATION_ITEM()
RATIONAL_B_SPLINE_SURFACE(((1.,0.708394529056577,1.00061746385311),(1.,
0.708058564167112,1.0006181752464),(1.,0.707430835372313,1.00061950443902),
(1.,0.70679668588064,1.00062084722723)))
REPRESENTATION_ITEM('')
SURFACE()
);
#3189=(
BOUNDED_SURFACE()
B_SPLINE_SURFACE(3,2,((#209837,#209838,#209839),(#209840,#209841,#209842),
(#209843,#209844,#209845),(#209846,#209847,#209848)),.UNSPECIFIED.,.F.,
 .F.,.F.)
B_SPLINE_SURFACE_WITH_KNOTS((4,4),(3,3),(-6.53231808922516E-18,0.000397394465448313),
(0.,1.),.UNSPECIFIED.)
GEOMETRIC_REPRESENTATION_ITEM()
RATIONAL_B_SPLINE_SURFACE(((1.,0.705498956110761,1.),(1.,0.705821764811792,
1.),(1.,0.706461952521145,1.),(1.,0.70710678118654,1.)))
REPRESENTATION_ITEM('')
SURFACE()
);
#3190=(
BOUNDED_SURFACE()
B_SPLINE_SURFACE(3,2,((#209854,#209855,#209856),(#209857,#209858,#209859),
(#209860,#209861,#209862),(#209863,#209864,#209865)),.UNSPECIFIED.,.F.,
 .F.,.F.)
B_SPLINE_SURFACE_WITH_KNOTS((4,4),(3,3),(0.,0.000397394410828728),(0.,1.),
 .UNSPECIFIED.)
GEOMETRIC_REPRESENTATION_ITEM()
RATIONAL_B_SPLINE_SURFACE(((1.,0.708689770883319,1.),(1.,0.708376440034518,
1.),(1.,0.707750498698381,1.),(1.,0.707106781186553,1.)))
REPRESENTATION_ITEM('')
SURFACE()
);
#3191=(
BOUNDED_SURFACE()
B_SPLINE_SURFACE(3,2,((#209871,#209872,#209873),(#209874,#209875,#209876),
(#209877,#209878,#209879),(#209880,#209881,#209882)),.UNSPECIFIED.,.F.,
 .F.,.F.)
B_SPLINE_SURFACE_WITH_KNOTS((4,4),(3,3),(0.,0.000511815090126188),(0.,1.00105592270323),
 .UNSPECIFIED.)
GEOMETRIC_REPRESENTATION_ITEM()
RATIONAL_B_SPLINE_SURFACE(((1.,0.705266242717189,1.00062243213145),(1.,
0.705584085908845,1.00062176089576),(1.,0.706182089450181,1.00062049800473),
(1.,0.706797508587185,1.00061919833465)))
REPRESENTATION_ITEM('')
SURFACE()
);
#3192=(
BOUNDED_SURFACE()
B_SPLINE_SURFACE(3,2,((#209884,#209885,#209886),(#209887,#209888,#209889),
(#209890,#209891,#209892),(#209893,#209894,#209895)),.UNSPECIFIED.,.F.,
 .F.,.F.)
B_SPLINE_SURFACE_WITH_KNOTS((4,4),(3,3),(0.,0.000397394428086621),(0.,1.),
 .UNSPECIFIED.)
GEOMETRIC_REPRESENTATION_ITEM()
RATIONAL_B_SPLINE_SURFACE(((1.,0.707106781186553,1.),(1.,0.706459846759084,
1.),(1.,0.705820510737283,1.),(1.,0.705498956110755,1.)))
REPRESENTATION_ITEM('')
SURFACE()
);
#3193=(
BOUNDED_SURFACE()
B_SPLINE_SURFACE(3,2,((#209901,#209902,#209903),(#209904,#209905,#209906),
(#209907,#209908,#209909),(#209910,#209911,#209912),(#209913,#209914,#209915),
(#209916,#209917,#209918)),.UNSPECIFIED.,.F.,.F.,.F.)
B_SPLINE_SURFACE_WITH_KNOTS((4,2,4),(3,3),(-3.15773882736403E-18,0.000257953807872849,
0.0005159076157457),(0.,1.),.UNSPECIFIED.)
GEOMETRIC_REPRESENTATION_ITEM()
RATIONAL_B_SPLINE_SURFACE(((1.,0.874619707139386,1.),(1.,0.874834349679202,
1.),(1.,0.854686104157527,1.),(1.,0.792476597915401,1.),(1.,0.750887854594934,
1.),(1.,0.705585838031451,1.)))
REPRESENTATION_ITEM('')
SURFACE()
);
#3194=(
BOUNDED_SURFACE()
B_SPLINE_SURFACE(3,2,((#209924,#209925,#209926),(#209927,#209928,#209929),
(#209930,#209931,#209932),(#209933,#209934,#209935)),.UNSPECIFIED.,.F.,
 .F.,.F.)
B_SPLINE_SURFACE_WITH_KNOTS((4,4),(3,3),(0.,0.000511815437699157),(0.,1.00105881331785),
 .UNSPECIFIED.)
GEOMETRIC_REPRESENTATION_ITEM()
RATIONAL_B_SPLINE_SURFACE(((1.,0.706796661945761,1.00062089519834),(1.,
0.707430821224659,1.00061955228576),(1.,0.708058545830114,1.00061822299941),
(1.,0.70839450525216,1.00061751156279)))
REPRESENTATION_ITEM('')
SURFACE()
);
#3195=(
BOUNDED_SURFACE()
B_SPLINE_SURFACE(3,2,((#209937,#209938,#209939),(#209940,#209941,#209942),
(#209943,#209944,#209945),(#209946,#209947,#209948),(#209949,#209950,#209951),
(#209952,#209953,#209954)),.UNSPECIFIED.,.F.,.F.,.F.)
B_SPLINE_SURFACE_WITH_KNOTS((4,2,4),(3,3),(2.71050543121376E-20,0.00025691531753126,
0.00051383063506252),(0.,1.),.UNSPECIFIED.)
GEOMETRIC_REPRESENTATION_ITEM()
RATIONAL_B_SPLINE_SURFACE(((1.,0.705585838031445,1.),(1.,0.750902433542712,
1.),(1.,0.792329530082526,1.),(1.,0.854288401594204,1.),(1.,0.874998031125109,
1.),(1.,0.874619707139405,1.)))
REPRESENTATION_ITEM('')
SURFACE()
);
#3196=(
BOUNDED_SURFACE()
B_SPLINE_SURFACE(3,2,((#209960,#209961,#209962),(#209963,#209964,#209965),
(#209966,#209967,#209968),(#209969,#209970,#209971),(#209972,#209973,#209974),
(#209975,#209976,#209977)),.UNSPECIFIED.,.F.,.F.,.F.)
B_SPLINE_SURFACE_WITH_KNOTS((4,2,4),(3,3),(-5.77337656848531E-18,0.000256592814262153,
0.000513185628524312),(0.,1.),.UNSPECIFIED.)
GEOMETRIC_REPRESENTATION_ITEM()
RATIONAL_B_SPLINE_SURFACE(((1.,0.708712527163637,1.),(1.,0.753780902613617,
1.),(1.,0.794538995769177,1.),(1.,0.855070770331119,1.),(1.,0.875018427445295,
1.),(1.,0.874619707139396,1.)))
REPRESENTATION_ITEM('')
SURFACE()
);
#3197=(
BOUNDED_SURFACE()
B_SPLINE_SURFACE(3,2,((#209979,#209980,#209981),(#209982,#209983,#209984),
(#209985,#209986,#209987),(#209988,#209989,#209990)),.UNSPECIFIED.,.F.,
 .F.,.F.)
B_SPLINE_SURFACE_WITH_KNOTS((4,4),(3,3),(-7.58941520739853E-18,0.000511815072430402),
(0.,1.00105598365911),.UNSPECIFIED.)
GEOMETRIC_REPRESENTATION_ITEM()
RATIONAL_B_SPLINE_SURFACE(((1.,0.706797490733615,1.00061923411719),(1.,
0.706182062146498,1.00062053388226),(1.,0.705584062768905,1.0006217968374),
(1.,0.705266224770394,1.00062246810086)))
REPRESENTATION_ITEM('')
SURFACE()
);
#3198=(
BOUNDED_SURFACE()
B_SPLINE_SURFACE(3,2,((#209996,#209997,#209998),(#209999,#210000,#210001),
(#210002,#210003,#210004),(#210005,#210006,#210007),(#210008,#210009,#210010),
(#210011,#210012,#210013)),.UNSPECIFIED.,.F.,.F.,.F.)
B_SPLINE_SURFACE_WITH_KNOTS((4,2,4),(3,3),(-3.14418630020796E-18,0.000257652232350881,
0.000515304464701764),(0.,1.),.UNSPECIFIED.)
GEOMETRIC_REPRESENTATION_ITEM()
RATIONAL_B_SPLINE_SURFACE(((1.,0.874619707139394,1.),(1.,0.874861180431435,
1.),(1.,0.855455725919893,1.),(1.,0.794699358956221,1.),(1.,0.753768977787944,
1.),(1.,0.708712527163638,1.)))
REPRESENTATION_ITEM('')
SURFACE()
);
#3199=(
BOUNDED_SURFACE()
B_SPLINE_SURFACE(3,2,((#210019,#210020,#210021),(#210022,#210023,#210024),
(#210025,#210026,#210027),(#210028,#210029,#210030)),.UNSPECIFIED.,.F.,
 .F.,.F.)
B_SPLINE_SURFACE_WITH_KNOTS((4,4),(3,3),(-1.40675231879994E-17,0.000397394373651907),
(0.,1.),.UNSPECIFIED.)
GEOMETRIC_REPRESENTATION_ITEM()
RATIONAL_B_SPLINE_SURFACE(((1.,0.707106781186542,1.),(1.,0.707752587915892,
1.),(1.,0.708377654540694,1.),(1.,0.708689770883334,1.)))
REPRESENTATION_ITEM('')
SURFACE()
);
#3200=(
BOUNDED_SURFACE()
B_SPLINE_SURFACE(3,2,((#210032,#210033,#210034),(#210035,#210036,#210037),
(#210038,#210039,#210040),(#210041,#210042,#210043)),.UNSPECIFIED.,.F.,
 .F.,.F.)
B_SPLINE_SURFACE_WITH_KNOTS((4,4),(3,3),(-6.42389787197661E-18,0.00051181545647979),
(0.,1.00105873159698),.UNSPECIFIED.)
GEOMETRIC_REPRESENTATION_ITEM()
RATIONAL_B_SPLINE_SURFACE(((1.,0.708394529057203,1.00061746385188),(1.,
0.708058564167751,1.00061817524516),(1.,0.707430835372928,1.00061950443778),
(1.,0.70679668588125,1.00062084722599)))
REPRESENTATION_ITEM('')
SURFACE()
);
#3201=(
BOUNDED_SURFACE()
B_SPLINE_SURFACE(3,2,((#210049,#210050,#210051),(#210052,#210053,#210054),
(#210055,#210056,#210057),(#210058,#210059,#210060)),.UNSPECIFIED.,.F.,
 .F.,.F.)
B_SPLINE_SURFACE_WITH_KNOTS((4,4),(3,3),(0.,0.000397394465448308),(0.,1.),
 .UNSPECIFIED.)
GEOMETRIC_REPRESENTATION_ITEM()
RATIONAL_B_SPLINE_SURFACE(((1.,0.705498956110747,1.),(1.,0.705821764811728,
1.),(1.,0.706461952521178,1.),(1.,0.707106781186542,1.)))
REPRESENTATION_ITEM('')
SURFACE()
);
#3202=(
BOUNDED_SURFACE()
B_SPLINE_SURFACE(3,2,((#210066,#210067,#210068),(#210069,#210070,#210071),
(#210072,#210073,#210074),(#210075,#210076,#210077)),.UNSPECIFIED.,.F.,
 .F.,.F.)
B_SPLINE_SURFACE_WITH_KNOTS((4,4),(3,3),(0.,0.000397394410828749),(0.,1.),
 .UNSPECIFIED.)
GEOMETRIC_REPRESENTATION_ITEM()
RATIONAL_B_SPLINE_SURFACE(((1.,0.708689770883333,1.),(1.,0.708376440034485,
1.),(1.,0.707750498698427,1.),(1.,0.707106781186548,1.)))
REPRESENTATION_ITEM('')
SURFACE()
);
#3203=(
BOUNDED_SURFACE()
B_SPLINE_SURFACE(3,2,((#210083,#210084,#210085),(#210086,#210087,#210088),
(#210089,#210090,#210091),(#210092,#210093,#210094)),.UNSPECIFIED.,.F.,
 .F.,.F.)
B_SPLINE_SURFACE_WITH_KNOTS((4,4),(3,3),(0.,0.00051181509012617),(0.,1.00105592270455),
 .UNSPECIFIED.)
GEOMETRIC_REPRESENTATION_ITEM()
RATIONAL_B_SPLINE_SURFACE(((1.,0.705266242716791,1.00062243213223),(1.,
0.705584085908443,1.00062176089654),(1.,0.706182089449806,1.00062049800551),
(1.,0.706797508586792,1.00061919833543)))
REPRESENTATION_ITEM('')
SURFACE()
);
#3204=(
BOUNDED_SURFACE()
B_SPLINE_SURFACE(3,2,((#210096,#210097,#210098),(#210099,#210100,#210101),
(#210102,#210103,#210104),(#210105,#210106,#210107)),.UNSPECIFIED.,.F.,
 .F.,.F.)
B_SPLINE_SURFACE_WITH_KNOTS((4,4),(3,3),(0.,0.000397394428086618),(0.,1.),
 .UNSPECIFIED.)
GEOMETRIC_REPRESENTATION_ITEM()
RATIONAL_B_SPLINE_SURFACE(((1.,0.707106781186552,1.),(1.,0.706459846759076,
1.),(1.,0.705820510737295,1.),(1.,0.705498956110739,1.)))
REPRESENTATION_ITEM('')
SURFACE()
);
#3205=(
BOUNDED_SURFACE()
B_SPLINE_SURFACE(3,2,((#210113,#210114,#210115),(#210116,#210117,#210118),
(#210119,#210120,#210121),(#210122,#210123,#210124),(#210125,#210126,#210127),
(#210128,#210129,#210130)),.UNSPECIFIED.,.F.,.F.,.F.)
B_SPLINE_SURFACE_WITH_KNOTS((4,2,4),(3,3),(0.,0.000257953807872849,0.000515907615745698),
(0.,1.),.UNSPECIFIED.)
GEOMETRIC_REPRESENTATION_ITEM()
RATIONAL_B_SPLINE_SURFACE(((1.,0.874619707139397,1.),(1.,0.874834349678898,
1.),(1.,0.854686104157902,1.),(1.,0.792476597915046,1.),(1.,0.750887854595174,
1.),(1.,0.70558583803143,1.)))
REPRESENTATION_ITEM('')
SURFACE()
);
#3206=(
BOUNDED_SURFACE()
B_SPLINE_SURFACE(3,2,((#210136,#210137,#210138),(#210139,#210140,#210141),
(#210142,#210143,#210144),(#210145,#210146,#210147)),.UNSPECIFIED.,.F.,
 .F.,.F.)
B_SPLINE_SURFACE_WITH_KNOTS((4,4),(3,3),(0.,0.000511815437699145),(0.,1.0010588133135),
 .UNSPECIFIED.)
GEOMETRIC_REPRESENTATION_ITEM()
RATIONAL_B_SPLINE_SURFACE(((1.,0.706796661947034,1.00062089519579),(1.,
0.707430821225921,1.00061955228321),(1.,0.708058545831377,1.00061822299687),
(1.,0.708394505253416,1.00061751156026)))
REPRESENTATION_ITEM('')
SURFACE()
);
#3207=(
BOUNDED_SURFACE()
B_SPLINE_SURFACE(3,2,((#210149,#210150,#210151),(#210152,#210153,#210154),
(#210155,#210156,#210157),(#210158,#210159,#210160),(#210161,#210162,#210163),
(#210164,#210165,#210166)),.UNSPECIFIED.,.F.,.F.,.F.)
B_SPLINE_SURFACE_WITH_KNOTS((4,2,4),(3,3),(-6.31547765472806E-18,0.000256915317531251,
0.000513830635062508),(0.,1.),.UNSPECIFIED.)
GEOMETRIC_REPRESENTATION_ITEM()
RATIONAL_B_SPLINE_SURFACE(((1.,0.705585838031427,1.),(1.,0.750902433542642,
1.),(1.,0.792329530082651,1.),(1.,0.854288401594041,1.),(1.,0.874998031125251,
1.),(1.,0.874619707139387,1.)))
REPRESENTATION_ITEM('')
SURFACE()
);
#3208=(
BOUNDED_SURFACE()
B_SPLINE_SURFACE(3,2,((#210172,#210173,#210174),(#210175,#210176,#210177),
(#210178,#210179,#210180),(#210181,#210182,#210183),(#210184,#210185,#210186),
(#210187,#210188,#210189)),.UNSPECIFIED.,.F.,.F.,.F.)
B_SPLINE_SURFACE_WITH_KNOTS((4,2,4),(3,3),(0.,0.000256592814262157,0.000513185628524314),
(0.,1.),.UNSPECIFIED.)
GEOMETRIC_REPRESENTATION_ITEM()
RATIONAL_B_SPLINE_SURFACE(((1.,0.708712527163669,1.),(1.,0.75378090261303,
1.),(1.,0.794538995769939,1.),(1.,0.855070770330402,1.),(1.,0.875018427445837,
1.),(1.,0.874619707139389,1.)))
REPRESENTATION_ITEM('')
SURFACE()
);
#3209=(
BOUNDED_SURFACE()
B_SPLINE_SURFACE(3,2,((#210191,#210192,#210193),(#210194,#210195,#210196),
(#210197,#210198,#210199),(#210200,#210201,#210202)),.UNSPECIFIED.,.F.,
 .F.,.F.)
B_SPLINE_SURFACE_WITH_KNOTS((4,4),(3,3),(2.71050543121376E-20,0.000511815072430395),
(0.,1.00105598366028),.UNSPECIFIED.)
GEOMETRIC_REPRESENTATION_ITEM()
RATIONAL_B_SPLINE_SURFACE(((1.,0.706797490733269,1.00061923411788),(1.,
0.706182062146185,1.00062053388294),(1.,0.705584062768579,1.00062179683809),
(1.,0.705266224770014,1.00062246810155)))
REPRESENTATION_ITEM('')
SURFACE()
);
#3210=(
BOUNDED_SURFACE()
B_SPLINE_SURFACE(3,2,((#210208,#210209,#210210),(#210211,#210212,#210213),
(#210214,#210215,#210216),(#210217,#210218,#210219),(#210220,#210221,#210222),
(#210223,#210224,#210225)),.UNSPECIFIED.,.F.,.F.,.F.)
B_SPLINE_SURFACE_WITH_KNOTS((4,2,4),(3,3),(0.,0.000257652232350882,0.000515304464701763),
(0.,1.),.UNSPECIFIED.)
GEOMETRIC_REPRESENTATION_ITEM()
RATIONAL_B_SPLINE_SURFACE(((1.,0.874619707139388,1.),(1.,0.874861180430589,
1.),(1.,0.855455725921058,1.),(1.,0.794699358955073,1.),(1.,0.753768977788798,
1.),(1.,0.708712527163669,1.)))
REPRESENTATION_ITEM('')
SURFACE()
);
#3211=(
BOUNDED_SURFACE()
B_SPLINE_SURFACE(3,2,((#210231,#210232,#210233),(#210234,#210235,#210236),
(#210237,#210238,#210239),(#210240,#210241,#210242)),.UNSPECIFIED.,.F.,
 .F.,.F.)
B_SPLINE_SURFACE_WITH_KNOTS((4,4),(3,3),(0.,0.000397394373651931),(0.,1.),
 .UNSPECIFIED.)
GEOMETRIC_REPRESENTATION_ITEM()
RATIONAL_B_SPLINE_SURFACE(((1.,0.707106781186543,1.),(1.,0.707752587915884,
1.),(1.,0.708377654540689,1.),(1.,0.708689770883328,1.)))
REPRESENTATION_ITEM('')
SURFACE()
);
#3212=(
BOUNDED_SURFACE()
B_SPLINE_SURFACE(3,2,((#210244,#210245,#210246),(#210247,#210248,#210249),
(#210250,#210251,#210252),(#210253,#210254,#210255)),.UNSPECIFIED.,.F.,
 .F.,.F.)
B_SPLINE_SURFACE_WITH_KNOTS((4,4),(3,3),(0.,0.000511815456479789),(0.,1.00105873159931),
 .UNSPECIFIED.)
GEOMETRIC_REPRESENTATION_ITEM()
RATIONAL_B_SPLINE_SURFACE(((1.,0.708394529056513,1.00061746385324),(1.,
0.708058564167068,1.00061817524653),(1.,0.707430835372242,1.00061950443915),
(1.,0.706796685880566,1.00062084722736)))
REPRESENTATION_ITEM('')
SURFACE()
);
#3213=(
BOUNDED_SURFACE()
B_SPLINE_SURFACE(3,2,((#210261,#210262,#210263),(#210264,#210265,#210266),
(#210267,#210268,#210269),(#210270,#210271,#210272)),.UNSPECIFIED.,.F.,
 .F.,.F.)
B_SPLINE_SURFACE_WITH_KNOTS((4,4),(3,3),(0.,0.000397394465448298),(0.,1.),
 .UNSPECIFIED.)
GEOMETRIC_REPRESENTATION_ITEM()
RATIONAL_B_SPLINE_SURFACE(((1.,0.705498956110754,1.),(1.,0.705821764811777,
1.),(1.,0.70646195252115,1.),(1.,0.707106781186543,1.)))
REPRESENTATION_ITEM('')
SURFACE()
);
#3214=(
BOUNDED_SURFACE()
B_SPLINE_SURFACE(3,2,((#210278,#210279,#210280),(#210281,#210282,#210283),
(#210284,#210285,#210286),(#210287,#210288,#210289)),.UNSPECIFIED.,.F.,
 .F.,.F.)
B_SPLINE_SURFACE_WITH_KNOTS((4,4),(3,3),(0.,0.000397394410828728),(0.,1.),
 .UNSPECIFIED.)
GEOMETRIC_REPRESENTATION_ITEM()
RATIONAL_B_SPLINE_SURFACE(((1.,0.708689770883309,1.),(1.,0.708376440034508,
1.),(1.,0.707750498698397,1.),(1.,0.707106781186548,1.)))
REPRESENTATION_ITEM('')
SURFACE()
);
#3215=(
BOUNDED_SURFACE()
B_SPLINE_SURFACE(3,2,((#210295,#210296,#210297),(#210298,#210299,#210300),
(#210301,#210302,#210303),(#210304,#210305,#210306)),.UNSPECIFIED.,.F.,
 .F.,.F.)
B_SPLINE_SURFACE_WITH_KNOTS((4,4),(3,3),(0.,0.000511815090126182),(0.,1.00105592270654),
 .UNSPECIFIED.)
GEOMETRIC_REPRESENTATION_ITEM()
RATIONAL_B_SPLINE_SURFACE(((1.,0.705266242716211,1.0006224321334),(1.,0.705584085907866,
1.00062176089771),(1.,0.706182089449231,1.00062049800668),(1.,0.706797508586209,
1.0006191983366)))
REPRESENTATION_ITEM('')
SURFACE()
);
#3216=(
BOUNDED_SURFACE()
B_SPLINE_SURFACE(3,2,((#210308,#210309,#210310),(#210311,#210312,#210313),
(#210314,#210315,#210316),(#210317,#210318,#210319)),.UNSPECIFIED.,.F.,
 .F.,.F.)
B_SPLINE_SURFACE_WITH_KNOTS((4,4),(3,3),(0.,0.00039739442808663),(0.,1.),
 .UNSPECIFIED.)
GEOMETRIC_REPRESENTATION_ITEM()
RATIONAL_B_SPLINE_SURFACE(((1.,0.70710678118655,1.),(1.,0.706459846759094,
1.),(1.,0.705820510737275,1.),(1.,0.705498956110756,1.)))
REPRESENTATION_ITEM('')
SURFACE()
);
#3217=(
BOUNDED_SURFACE()
B_SPLINE_SURFACE(3,2,((#210325,#210326,#210327),(#210328,#210329,#210330),
(#210331,#210332,#210333),(#210334,#210335,#210336),(#210337,#210338,#210339),
(#210340,#210341,#210342)),.UNSPECIFIED.,.F.,.F.,.F.)
B_SPLINE_SURFACE_WITH_KNOTS((4,2,4),(3,3),(0.,0.000257953807872841,0.000515907615745682),
(0.,1.),.UNSPECIFIED.)
GEOMETRIC_REPRESENTATION_ITEM()
RATIONAL_B_SPLINE_SURFACE(((1.,0.874619707139387,1.),(1.,0.874834349678916,
1.),(1.,0.854686104157876,1.),(1.,0.79247659791507,1.),(1.,0.750887854595179,
1.),(1.,0.705585838031445,1.)))
REPRESENTATION_ITEM('')
SURFACE()
);
#3218=(
BOUNDED_SURFACE()
B_SPLINE_SURFACE(3,2,((#210348,#210349,#210350),(#210351,#210352,#210353),
(#210354,#210355,#210356),(#210357,#210358,#210359)),.UNSPECIFIED.,.F.,
 .F.,.F.)
B_SPLINE_SURFACE_WITH_KNOTS((4,4),(3,3),(-6.91178884959509E-18,0.000511815437699147),
(0.,1.00105881331641),.UNSPECIFIED.)
GEOMETRIC_REPRESENTATION_ITEM()
RATIONAL_B_SPLINE_SURFACE(((1.,0.70679666194618,1.00062089519749),(1.,0.707430821225043,
1.00061955228491),(1.,0.708058545830579,1.00061822299857),(1.,0.708394505252563,
1.00061751156195)))
REPRESENTATION_ITEM('')
SURFACE()
);
#3219=(
BOUNDED_SURFACE()
B_SPLINE_SURFACE(3,2,((#210361,#210362,#210363),(#210364,#210365,#210366),
(#210367,#210368,#210369),(#210370,#210371,#210372),(#210373,#210374,#210375),
(#210376,#210377,#210378)),.UNSPECIFIED.,.F.,.F.,.F.)
B_SPLINE_SURFACE_WITH_KNOTS((4,2,4),(3,3),(-2.71050543121376E-20,0.000256915317531261,
0.000513830635062522),(0.,1.),.UNSPECIFIED.)
GEOMETRIC_REPRESENTATION_ITEM()
RATIONAL_B_SPLINE_SURFACE(((1.,0.705585838031456,1.),(1.,0.750902433542761,
1.),(1.,0.792329530082443,1.),(1.,0.854288401594255,1.),(1.,0.874998031125089,
1.),(1.,0.874619707139388,1.)))
REPRESENTATION_ITEM('')
SURFACE()
);
#3220=(
BOUNDED_SURFACE()
B_SPLINE_SURFACE(3,2,((#210384,#210385,#210386),(#210387,#210388,#210389),
(#210390,#210391,#210392),(#210393,#210394,#210395),(#210396,#210397,#210398),
(#210399,#210400,#210401)),.UNSPECIFIED.,.F.,.F.,.F.)
B_SPLINE_SURFACE_WITH_KNOTS((4,2,4),(3,3),(0.,0.000256592814262156,0.000513185628524312),
(0.,1.),.UNSPECIFIED.)
GEOMETRIC_REPRESENTATION_ITEM()
RATIONAL_B_SPLINE_SURFACE(((1.,0.70871252716368,1.),(1.,0.753780902613984,
1.),(1.,0.794538995768662,1.),(1.,0.855070770331644,1.),(1.,0.875018427444918,
1.),(1.,0.874619707139392,1.)))
REPRESENTATION_ITEM('')
SURFACE()
);
#3221=(
BOUNDED_SURFACE()
B_SPLINE_SURFACE(3,2,((#210403,#210404,#210405),(#210406,#210407,#210408),
(#210409,#210410,#210411),(#210412,#210413,#210414)),.UNSPECIFIED.,.F.,
 .F.,.F.)
B_SPLINE_SURFACE_WITH_KNOTS((4,4),(3,3),(0.,0.000511815072430398),(0.,1.00105598366037),
 .UNSPECIFIED.)
GEOMETRIC_REPRESENTATION_ITEM()
RATIONAL_B_SPLINE_SURFACE(((1.,0.706797490733248,1.00061923411793),(1.,
0.706182062146152,1.000620533883),(1.,0.705584062768531,1.00062179683814),
(1.,0.705266224770001,1.00062246810161)))
REPRESENTATION_ITEM('')
SURFACE()
);
#3222=(
BOUNDED_SURFACE()
B_SPLINE_SURFACE(3,2,((#210420,#210421,#210422),(#210423,#210424,#210425),
(#210426,#210427,#210428),(#210429,#210430,#210431),(#210432,#210433,#210434),
(#210435,#210436,#210437)),.UNSPECIFIED.,.F.,.F.,.F.)
B_SPLINE_SURFACE_WITH_KNOTS((4,2,4),(3,3),(-8.26704156520197E-19,0.000257652232350878,
0.000515304464701757),(0.,1.),.UNSPECIFIED.)
GEOMETRIC_REPRESENTATION_ITEM()
RATIONAL_B_SPLINE_SURFACE(((1.,0.87461970713939,1.),(1.,0.874861180431015,
1.),(1.,0.855455725920467,1.),(1.,0.794699358955663,1.),(1.,0.753768977788366,
1.),(1.,0.708712527163666,1.)))
REPRESENTATION_ITEM('')
SURFACE()
);
#3223=(
BOUNDED_SURFACE()
B_SPLINE_SURFACE(3,2,((#210443,#210444,#210445),(#210446,#210447,#210448),
(#210449,#210450,#210451),(#210452,#210453,#210454)),.UNSPECIFIED.,.F.,
 .F.,.F.)
B_SPLINE_SURFACE_WITH_KNOTS((4,4),(3,3),(0.,0.000397394373651932),(0.,1.),
 .UNSPECIFIED.)
GEOMETRIC_REPRESENTATION_ITEM()
RATIONAL_B_SPLINE_SURFACE(((1.,0.707106781186547,1.),(1.,0.707752587915898,
1.),(1.,0.708377654540681,1.),(1.,0.708689770883335,1.)))
REPRESENTATION_ITEM('')
SURFACE()
);
#3224=(
BOUNDED_SURFACE()
B_SPLINE_SURFACE(3,2,((#210456,#210457,#210458),(#210459,#210460,#210461),
(#210462,#210463,#210464),(#210465,#210466,#210467)),.UNSPECIFIED.,.F.,
 .F.,.F.)
B_SPLINE_SURFACE_WITH_KNOTS((4,4),(3,3),(0.,0.000511815456479785),(0.,1.00105873159947),
 .UNSPECIFIED.)
GEOMETRIC_REPRESENTATION_ITEM()
RATIONAL_B_SPLINE_SURFACE(((1.,0.708394529056471,1.00061746385333),(1.,
0.708058564167021,1.00061817524662),(1.,0.70743083537221,1.00061950443924),
(1.,0.70679668588052,1.00062084722745)))
REPRESENTATION_ITEM('')
SURFACE()
);
#3225=(
BOUNDED_SURFACE()
B_SPLINE_SURFACE(3,2,((#210473,#210474,#210475),(#210476,#210477,#210478),
(#210479,#210480,#210481),(#210482,#210483,#210484)),.UNSPECIFIED.,.F.,
 .F.,.F.)
B_SPLINE_SURFACE_WITH_KNOTS((4,4),(3,3),(0.,0.000397394465448308),(0.,1.),
 .UNSPECIFIED.)
GEOMETRIC_REPRESENTATION_ITEM()
RATIONAL_B_SPLINE_SURFACE(((1.,0.705498956110727,1.),(1.,0.705821764811783,
1.),(1.,0.706461952521138,1.),(1.,0.707106781186548,1.)))
REPRESENTATION_ITEM('')
SURFACE()
);
#3226=(
BOUNDED_SURFACE()
B_SPLINE_SURFACE(3,2,((#225174,#225175,#225176),(#225177,#225178,#225179),
(#225180,#225181,#225182),(#225183,#225184,#225185)),.UNSPECIFIED.,.F.,
 .F.,.F.)
B_SPLINE_SURFACE_WITH_KNOTS((4,4),(3,3),(0.,0.00039739441082874),(0.,1.),
 .UNSPECIFIED.)
GEOMETRIC_REPRESENTATION_ITEM()
RATIONAL_B_SPLINE_SURFACE(((1.,0.708689770883314,1.),(1.,0.708376440034511,
1.),(1.,0.707750498698406,1.),(1.,0.707106781186548,1.)))
REPRESENTATION_ITEM('')
SURFACE()
);
#3227=(
BOUNDED_SURFACE()
B_SPLINE_SURFACE(3,2,((#225191,#225192,#225193),(#225194,#225195,#225196),
(#225197,#225198,#225199),(#225200,#225201,#225202)),.UNSPECIFIED.,.F.,
 .F.,.F.)
B_SPLINE_SURFACE_WITH_KNOTS((4,4),(3,3),(0.,0.000511815090126175),(0.,1.00105592270397),
 .UNSPECIFIED.)
GEOMETRIC_REPRESENTATION_ITEM()
RATIONAL_B_SPLINE_SURFACE(((1.,0.705266242716963,1.00062243213188),(1.,
0.70558408590863,1.0006217608962),(1.,0.706182089449966,1.00062049800517),
(1.,0.706797508586963,1.00061919833509)))
REPRESENTATION_ITEM('')
SURFACE()
);
#3228=(
BOUNDED_SURFACE()
B_SPLINE_SURFACE(3,2,((#225204,#225205,#225206),(#225207,#225208,#225209),
(#225210,#225211,#225212),(#225213,#225214,#225215)),.UNSPECIFIED.,.F.,
 .F.,.F.)
B_SPLINE_SURFACE_WITH_KNOTS((4,4),(3,3),(-7.07441917546792E-18,0.000397394428086617),
(0.,1.),.UNSPECIFIED.)
GEOMETRIC_REPRESENTATION_ITEM()
RATIONAL_B_SPLINE_SURFACE(((1.,0.707106781186548,1.),(1.,0.706459846759103,
1.),(1.,0.705820510737259,1.),(1.,0.705498956110752,1.)))
REPRESENTATION_ITEM('')
SURFACE()
);
#3229=(
BOUNDED_SURFACE()
B_SPLINE_SURFACE(3,2,((#225221,#225222,#225223),(#225224,#225225,#225226),
(#225227,#225228,#225229),(#225230,#225231,#225232),(#225233,#225234,#225235),
(#225236,#225237,#225238)),.UNSPECIFIED.,.F.,.F.,.F.)
B_SPLINE_SURFACE_WITH_KNOTS((4,2,4),(3,3),(9.48676900924816E-20,0.000257953807872846,
0.000515907615745692),(0.,1.),.UNSPECIFIED.)
GEOMETRIC_REPRESENTATION_ITEM()
RATIONAL_B_SPLINE_SURFACE(((1.,0.874619707139395,1.),(1.,0.874834349678943,
1.),(1.,0.854686104157858,1.),(1.,0.79247659791508,1.),(1.,0.750887854595179,
1.),(1.,0.705585838031436,1.)))
REPRESENTATION_ITEM('')
SURFACE()
);
#3230=(
BOUNDED_SURFACE()
B_SPLINE_SURFACE(3,2,((#225244,#225245,#225246),(#225247,#225248,#225249),
(#225250,#225251,#225252),(#225253,#225254,#225255)),.UNSPECIFIED.,.F.,
 .F.,.F.)
B_SPLINE_SURFACE_WITH_KNOTS((4,4),(3,3),(0.,0.000511815437699145),(0.,1.00105881331503),
 .UNSPECIFIED.)
GEOMETRIC_REPRESENTATION_ITEM()
RATIONAL_B_SPLINE_SURFACE(((1.,0.706796661946587,1.00062089519668),(1.,
0.707430821225455,1.00061955228411),(1.,0.708058545830982,1.00061822299776),
(1.,0.708394505252967,1.00061751156115)))
REPRESENTATION_ITEM('')
SURFACE()
);
#3231=(
BOUNDED_SURFACE()
B_SPLINE_SURFACE(3,2,((#225257,#225258,#225259),(#225260,#225261,#225262),
(#225263,#225264,#225265),(#225266,#225267,#225268),(#225269,#225270,#225271),
(#225272,#225273,#225274)),.UNSPECIFIED.,.F.,.F.,.F.)
B_SPLINE_SURFACE_WITH_KNOTS((4,2,4),(3,3),(-1.62630325872826E-19,0.000256915317531258,
0.000513830635062517),(0.,1.),.UNSPECIFIED.)
GEOMETRIC_REPRESENTATION_ITEM()
RATIONAL_B_SPLINE_SURFACE(((1.,0.705585838031442,1.),(1.,0.750902433542864,
1.),(1.,0.792329530082365,1.),(1.,0.854288401594348,1.),(1.,0.874998031125021,
1.),(1.,0.874619707139395,1.)))
REPRESENTATION_ITEM('')
SURFACE()
);
#3232=(
BOUNDED_SURFACE()
B_SPLINE_SURFACE(3,2,((#225280,#225281,#225282),(#225283,#225284,#225285),
(#225286,#225287,#225288),(#225289,#225290,#225291),(#225292,#225293,#225294),
(#225295,#225296,#225297)),.UNSPECIFIED.,.F.,.F.,.F.)
B_SPLINE_SURFACE_WITH_KNOTS((4,2,4),(3,3),(-2.49366499671666E-18,0.000256592814262156,
0.000513185628524314),(0.,1.),.UNSPECIFIED.)
GEOMETRIC_REPRESENTATION_ITEM()
RATIONAL_B_SPLINE_SURFACE(((1.,0.708712527163662,1.),(1.,0.753780902613589,
1.),(1.,0.794538995769203,1.),(1.,0.855070770331116,1.),(1.,0.875018427445322,
1.),(1.,0.8746197071394,1.)))
REPRESENTATION_ITEM('')
SURFACE()
);
#3233=(
BOUNDED_SURFACE()
B_SPLINE_SURFACE(3,2,((#225299,#225300,#225301),(#225302,#225303,#225304),
(#225305,#225306,#225307),(#225308,#225309,#225310)),.UNSPECIFIED.,.F.,
 .F.,.F.)
B_SPLINE_SURFACE_WITH_KNOTS((4,4),(3,3),(2.71050543121376E-20,0.000511815072430401),
(0.,1.00105598366065),.UNSPECIFIED.)
GEOMETRIC_REPRESENTATION_ITEM()
RATIONAL_B_SPLINE_SURFACE(((1.,0.706797490733166,1.00061923411809),(1.,
0.706182062146078,1.00062053388316),(1.,0.705584062768454,1.0006217968383),
(1.,0.705266224769923,1.00062246810177)))
REPRESENTATION_ITEM('')
SURFACE()
);
#3234=(
BOUNDED_SURFACE()
B_SPLINE_SURFACE(3,2,((#225316,#225317,#225318),(#225319,#225320,#225321),
(#225322,#225323,#225324),(#225325,#225326,#225327),(#225328,#225329,#225330),
(#225331,#225332,#225333)),.UNSPECIFIED.,.F.,.F.,.F.)
B_SPLINE_SURFACE_WITH_KNOTS((4,2,4),(3,3),(-9.48676900924816E-20,0.00025765223235088,
0.000515304464701759),(0.,1.),.UNSPECIFIED.)
GEOMETRIC_REPRESENTATION_ITEM()
RATIONAL_B_SPLINE_SURFACE(((1.,0.874619707139394,1.),(1.,0.874861180430754,
1.),(1.,0.855455725920805,1.),(1.,0.794699358955339,1.),(1.,0.753768977788591,
1.),(1.,0.708712527163663,1.)))
REPRESENTATION_ITEM('')
SURFACE()
);
#3235=(
BOUNDED_SURFACE()
B_SPLINE_SURFACE(3,2,((#225339,#225340,#225341),(#225342,#225343,#225344),
(#225345,#225346,#225347),(#225348,#225349,#225350)),.UNSPECIFIED.,.F.,
 .F.,.F.)
B_SPLINE_SURFACE_WITH_KNOTS((4,4),(3,3),(0.,0.000397394373651912),(0.,1.),
 .UNSPECIFIED.)
GEOMETRIC_REPRESENTATION_ITEM()
RATIONAL_B_SPLINE_SURFACE(((1.,0.707106781186548,1.),(1.,0.707752587915877,
1.),(1.,0.708377654540693,1.),(1.,0.708689770883314,1.)))
REPRESENTATION_ITEM('')
SURFACE()
);
#3236=(
BOUNDED_SURFACE()
B_SPLINE_SURFACE(3,2,((#225352,#225353,#225354),(#225355,#225356,#225357),
(#225358,#225359,#225360),(#225361,#225362,#225363)),.UNSPECIFIED.,.F.,
 .F.,.F.)
B_SPLINE_SURFACE_WITH_KNOTS((4,4),(3,3),(-5.61074624261249E-18,0.000511815456479793),
(0.,1.00105873159934),.UNSPECIFIED.)
GEOMETRIC_REPRESENTATION_ITEM()
RATIONAL_B_SPLINE_SURFACE(((1.,0.708394529056523,1.00061746385326),(1.,
0.70805856416705,1.00061817524655),(1.,0.70743083537224,1.00061950443917),
(1.,0.706796685880558,1.00062084722738)))
REPRESENTATION_ITEM('')
SURFACE()
);
#3237=(
BOUNDED_SURFACE()
B_SPLINE_SURFACE(3,2,((#225369,#225370,#225371),(#225372,#225373,#225374),
(#225375,#225376,#225377),(#225378,#225379,#225380)),.UNSPECIFIED.,.F.,
 .F.,.F.)
B_SPLINE_SURFACE_WITH_KNOTS((4,4),(3,3),(0.,0.000397394465448316),(0.,1.),
 .UNSPECIFIED.)
GEOMETRIC_REPRESENTATION_ITEM()
RATIONAL_B_SPLINE_SURFACE(((1.,0.705498956110752,1.),(1.,0.705821764811793,
1.),(1.,0.70646195252114,1.),(1.,0.707106781186548,1.)))
REPRESENTATION_ITEM('')
SURFACE()
);
#3238=(
BOUNDED_SURFACE()
B_SPLINE_SURFACE(3,2,((#240891,#240892,#240893),(#240894,#240895,#240896),
(#240897,#240898,#240899),(#240900,#240901,#240902)),.UNSPECIFIED.,.F.,
 .F.,.F.)
B_SPLINE_SURFACE_WITH_KNOTS((4,4),(3,3),(-2.71050543121376E-20,0.000397394410828744),
(0.,1.),.UNSPECIFIED.)
GEOMETRIC_REPRESENTATION_ITEM()
RATIONAL_B_SPLINE_SURFACE(((1.,0.708689770883338,1.),(1.,0.708376440034495,
1.),(1.,0.707750498698416,1.),(1.,0.707106781186545,1.)))
REPRESENTATION_ITEM('')
SURFACE()
);
#3239=(
BOUNDED_SURFACE()
B_SPLINE_SURFACE(3,2,((#240908,#240909,#240910),(#240911,#240912,#240913),
(#240914,#240915,#240916),(#240917,#240918,#240919)),.UNSPECIFIED.,.F.,
 .F.,.F.)
B_SPLINE_SURFACE_WITH_KNOTS((4,4),(3,3),(2.71050543121376E-20,0.000511815090126173),
(0.,1.00105592270292),.UNSPECIFIED.)
GEOMETRIC_REPRESENTATION_ITEM()
RATIONAL_B_SPLINE_SURFACE(((1.,0.705266242717266,1.00062243213126),(1.,
0.705584085908932,1.00062176089558),(1.,0.706182089450283,1.00062049800455),
(1.,0.706797508587271,1.00061919833447)))
REPRESENTATION_ITEM('')
SURFACE()
);
#3240=(
BOUNDED_SURFACE()
B_SPLINE_SURFACE(3,2,((#240921,#240922,#240923),(#240924,#240925,#240926),
(#240927,#240928,#240929),(#240930,#240931,#240932)),.UNSPECIFIED.,.F.,
 .F.,.F.)
B_SPLINE_SURFACE_WITH_KNOTS((4,4),(3,3),(-8.13151629364128E-20,0.00039739442808662),
(0.,1.),.UNSPECIFIED.)
GEOMETRIC_REPRESENTATION_ITEM()
RATIONAL_B_SPLINE_SURFACE(((1.,0.70710678118655,1.),(1.,0.706459846759071,
1.),(1.,0.705820510737309,1.),(1.,0.705498956110743,1.)))
REPRESENTATION_ITEM('')
SURFACE()
);
#3241=(
BOUNDED_SURFACE()
B_SPLINE_SURFACE(3,2,((#240938,#240939,#240940),(#240941,#240942,#240943),
(#240944,#240945,#240946),(#240947,#240948,#240949),(#240950,#240951,#240952),
(#240953,#240954,#240955)),.UNSPECIFIED.,.F.,.F.,.F.)
B_SPLINE_SURFACE_WITH_KNOTS((4,2,4),(3,3),(0.,0.00025795380787285,0.0005159076157457),
(0.,1.),.UNSPECIFIED.)
GEOMETRIC_REPRESENTATION_ITEM()
RATIONAL_B_SPLINE_SURFACE(((1.,0.87461970713939,1.),(1.,0.874834349679194,
1.),(1.,0.854686104157516,1.),(1.,0.792476597915439,1.),(1.,0.750887854594908,
1.),(1.,0.705585838031442,1.)))
REPRESENTATION_ITEM('')
SURFACE()
);
#3242=(
BOUNDED_SURFACE()
B_SPLINE_SURFACE(3,2,((#240961,#240962,#240963),(#240964,#240965,#240966),
(#240967,#240968,#240969),(#240970,#240971,#240972)),.UNSPECIFIED.,.F.,
 .F.,.F.)
B_SPLINE_SURFACE_WITH_KNOTS((4,4),(3,3),(8.13151629364128E-20,0.000511815437699155),
(0.,1.001058813318),.UNSPECIFIED.)
GEOMETRIC_REPRESENTATION_ITEM()
RATIONAL_B_SPLINE_SURFACE(((1.,0.706796661945717,1.00062089519843),(1.,
0.707430821224596,1.00061955228585),(1.,0.708058545830099,1.0006182229995),
(1.,0.708394505252105,1.00061751156288)))
REPRESENTATION_ITEM('')
SURFACE()
);
#3243=(
BOUNDED_SURFACE()
B_SPLINE_SURFACE(3,2,((#240974,#240975,#240976),(#240977,#240978,#240979),
(#240980,#240981,#240982),(#240983,#240984,#240985),(#240986,#240987,#240988),
(#240989,#240990,#240991)),.UNSPECIFIED.,.F.,.F.,.F.)
B_SPLINE_SURFACE_WITH_KNOTS((4,2,4),(3,3),(-1.0842021724855E-19,0.000256915317531264,
0.000513830635062529),(0.,1.),.UNSPECIFIED.)
GEOMETRIC_REPRESENTATION_ITEM()
RATIONAL_B_SPLINE_SURFACE(((1.,0.705585838031443,1.),(1.,0.750902433543475,
1.),(1.,0.792329530081552,1.),(1.,0.85428840159518,1.),(1.,0.874998031124423,
1.),(1.,0.87461970713939,1.)))
REPRESENTATION_ITEM('')
SURFACE()
);
#3244=(
BOUNDED_SURFACE()
B_SPLINE_SURFACE(3,2,((#240997,#240998,#240999),(#241000,#241001,#241002),
(#241003,#241004,#241005),(#241006,#241007,#241008),(#241009,#241010,#241011),
(#241012,#241013,#241014)),.UNSPECIFIED.,.F.,.F.,.F.)
B_SPLINE_SURFACE_WITH_KNOTS((4,2,4),(3,3),(1.0842021724855E-19,0.000256592814262158,
0.000513185628524316),(0.,1.),.UNSPECIFIED.)
GEOMETRIC_REPRESENTATION_ITEM()
RATIONAL_B_SPLINE_SURFACE(((1.,0.708712527163671,1.),(1.,0.753780902613763,
1.),(1.,0.794538995768961,1.),(1.,0.855070770331352,1.),(1.,0.875018427445139,
1.),(1.,0.874619707139394,1.)))
REPRESENTATION_ITEM('')
SURFACE()
);
#3245=(
BOUNDED_SURFACE()
B_SPLINE_SURFACE(3,2,((#241016,#241017,#241018),(#241019,#241020,#241021),
(#241022,#241023,#241024),(#241025,#241026,#241027)),.UNSPECIFIED.,.F.,
 .F.,.F.)
B_SPLINE_SURFACE_WITH_KNOTS((4,4),(3,3),(4.87890977618477E-19,0.000511815072430394),
(0.,1.00105598365812),.UNSPECIFIED.)
GEOMETRIC_REPRESENTATION_ITEM()
RATIONAL_B_SPLINE_SURFACE(((1.,0.706797490733907,1.00061923411661),(1.,
0.706182062146832,1.00062053388167),(1.,0.705584062769189,1.00062179683681),
(1.,0.705266224770674,1.00062246810027)))
REPRESENTATION_ITEM('')
SURFACE()
);
#3246=(
BOUNDED_SURFACE()
B_SPLINE_SURFACE(3,2,((#241033,#241034,#241035),(#241036,#241037,#241038),
(#241039,#241040,#241041),(#241042,#241043,#241044),(#241045,#241046,#241047),
(#241048,#241049,#241050)),.UNSPECIFIED.,.F.,.F.,.F.)
B_SPLINE_SURFACE_WITH_KNOTS((4,2,4),(3,3),(1.35525271560688E-20,0.000257652232350882,
0.000515304464701764),(0.,1.),.UNSPECIFIED.)
GEOMETRIC_REPRESENTATION_ITEM()
RATIONAL_B_SPLINE_SURFACE(((1.,0.874619707139383,1.),(1.,0.874861180430713,
1.),(1.,0.85545572592086,1.),(1.,0.794699358955259,1.),(1.,0.753768977788642,
1.),(1.,0.708712527163656,1.)))
REPRESENTATION_ITEM('')
SURFACE()
);
#3247=(
BOUNDED_SURFACE()
B_SPLINE_SURFACE(3,2,((#241056,#241057,#241058),(#241059,#241060,#241061),
(#241062,#241063,#241064),(#241065,#241066,#241067)),.UNSPECIFIED.,.F.,
 .F.,.F.)
B_SPLINE_SURFACE_WITH_KNOTS((4,4),(3,3),(8.13151629364128E-20,0.000397394373651917),
(0.,1.),.UNSPECIFIED.)
GEOMETRIC_REPRESENTATION_ITEM()
RATIONAL_B_SPLINE_SURFACE(((1.,0.707106781186548,1.),(1.,0.707752587915901,
1.),(1.,0.708377654540656,1.),(1.,0.708689770883324,1.)))
REPRESENTATION_ITEM('')
SURFACE()
);
#3248=(
BOUNDED_SURFACE()
B_SPLINE_SURFACE(3,2,((#241069,#241070,#241071),(#241072,#241073,#241074),
(#241075,#241076,#241077),(#241078,#241079,#241080)),.UNSPECIFIED.,.F.,
 .F.,.F.)
B_SPLINE_SURFACE_WITH_KNOTS((4,4),(3,3),(-2.71050543121376E-20,0.000511815456479787),
(0.,1.00105873159928),.UNSPECIFIED.)
GEOMETRIC_REPRESENTATION_ITEM()
RATIONAL_B_SPLINE_SURFACE(((1.,0.708394529056518,1.00061746385322),(1.,
0.708058564167046,1.00061817524651),(1.,0.707430835372269,1.00061950443913),
(1.,0.706796685880576,1.00062084722735)))
REPRESENTATION_ITEM('')
SURFACE()
);
#3249=(
BOUNDED_SURFACE()
B_SPLINE_SURFACE(3,2,((#241086,#241087,#241088),(#241089,#241090,#241091),
(#241092,#241093,#241094),(#241095,#241096,#241097)),.UNSPECIFIED.,.F.,
 .F.,.F.)
B_SPLINE_SURFACE_WITH_KNOTS((4,4),(3,3),(2.71050543121376E-20,0.000397394465448306),
(0.,1.),.UNSPECIFIED.)
GEOMETRIC_REPRESENTATION_ITEM()
RATIONAL_B_SPLINE_SURFACE(((1.,0.705498956110759,1.),(1.,0.70582176481179,
1.),(1.,0.706461952521145,1.),(1.,0.707106781186548,1.)))
REPRESENTATION_ITEM('')
SURFACE()
);
#3250=(
BOUNDED_SURFACE()
B_SPLINE_SURFACE(3,2,((#241103,#241104,#241105),(#241106,#241107,#241108),
(#241109,#241110,#241111),(#241112,#241113,#241114)),.UNSPECIFIED.,.F.,
 .F.,.F.)
B_SPLINE_SURFACE_WITH_KNOTS((4,4),(3,3),(0.,0.000397394410828732),(0.,1.),
 .UNSPECIFIED.)
GEOMETRIC_REPRESENTATION_ITEM()
RATIONAL_B_SPLINE_SURFACE(((1.,0.708689770883319,1.),(1.,0.70837644003452,
1.),(1.,0.70775049869839,1.),(1.,0.70710678118655,1.)))
REPRESENTATION_ITEM('')
SURFACE()
);
#3251=(
BOUNDED_SURFACE()
B_SPLINE_SURFACE(3,2,((#241120,#241121,#241122),(#241123,#241124,#241125),
(#241126,#241127,#241128),(#241129,#241130,#241131)),.UNSPECIFIED.,.F.,
 .F.,.F.)
B_SPLINE_SURFACE_WITH_KNOTS((4,4),(3,3),(1.35525271560688E-19,0.000511815090126187),
(0.,1.00105592270021),.UNSPECIFIED.)
GEOMETRIC_REPRESENTATION_ITEM()
RATIONAL_B_SPLINE_SURFACE(((1.,0.705266242718048,1.00062243212966),(1.,
0.705584085909746,1.00062176089398),(1.,0.706182089451072,1.00062049800295),
(1.,0.706797508588059,1.00061919833288)))
REPRESENTATION_ITEM('')
SURFACE()
);
#3252=(
BOUNDED_SURFACE()
B_SPLINE_SURFACE(3,2,((#241133,#241134,#241135),(#241136,#241137,#241138),
(#241139,#241140,#241141),(#241142,#241143,#241144)),.UNSPECIFIED.,.F.,
 .F.,.F.)
B_SPLINE_SURFACE_WITH_KNOTS((4,4),(3,3),(0.,0.000397394428086623),(0.,1.),
 .UNSPECIFIED.)
GEOMETRIC_REPRESENTATION_ITEM()
RATIONAL_B_SPLINE_SURFACE(((1.,0.707106781186546,1.),(1.,0.706459846759076,
1.),(1.,0.705820510737292,1.),(1.,0.705498956110753,1.)))
REPRESENTATION_ITEM('')
SURFACE()
);
#3253=(
BOUNDED_SURFACE()
B_SPLINE_SURFACE(3,2,((#241150,#241151,#241152),(#241153,#241154,#241155),
(#241156,#241157,#241158),(#241159,#241160,#241161),(#241162,#241163,#241164),
(#241165,#241166,#241167)),.UNSPECIFIED.,.F.,.F.,.F.)
B_SPLINE_SURFACE_WITH_KNOTS((4,2,4),(3,3),(0.,0.000257953807872846,0.000515907615745692),
(0.,1.),.UNSPECIFIED.)
GEOMETRIC_REPRESENTATION_ITEM()
RATIONAL_B_SPLINE_SURFACE(((1.,0.874619707139395,1.),(1.,0.874834349679043,
1.),(1.,0.854686104157736,1.),(1.,0.792476597915218,1.),(1.,0.750887854595055,
1.),(1.,0.705585838031455,1.)))
REPRESENTATION_ITEM('')
SURFACE()
);
#3254=(
BOUNDED_SURFACE()
B_SPLINE_SURFACE(3,2,((#241173,#241174,#241175),(#241176,#241177,#241178),
(#241179,#241180,#241181),(#241182,#241183,#241184)),.UNSPECIFIED.,.F.,
 .F.,.F.)
B_SPLINE_SURFACE_WITH_KNOTS((4,4),(3,3),(0.,0.000511815437699164),(0.,1.00105881331854),
 .UNSPECIFIED.)
GEOMETRIC_REPRESENTATION_ITEM()
RATIONAL_B_SPLINE_SURFACE(((1.,0.706796661945554,1.00062089519875),(1.,
0.707430821224427,1.00061955228617),(1.,0.708058545829957,1.00061822299982),
(1.,0.708394505251943,1.0006175115632)))
REPRESENTATION_ITEM('')
SURFACE()
);
#3255=(
BOUNDED_SURFACE()
B_SPLINE_SURFACE(3,2,((#241186,#241187,#241188),(#241189,#241190,#241191),
(#241192,#241193,#241194),(#241195,#241196,#241197),(#241198,#241199,#241200),
(#241201,#241202,#241203)),.UNSPECIFIED.,.F.,.F.,.F.)
B_SPLINE_SURFACE_WITH_KNOTS((4,2,4),(3,3),(0.,0.000256915317531264,0.000513830635062528),
(0.,1.),.UNSPECIFIED.)
GEOMETRIC_REPRESENTATION_ITEM()
RATIONAL_B_SPLINE_SURFACE(((1.,0.70558583803145,1.),(1.,0.75090243354219,
1.),(1.,0.792329530083307,1.),(1.,0.854288401593428,1.),(1.,0.874998031125737,
1.),(1.,0.874619707139414,1.)))
REPRESENTATION_ITEM('')
SURFACE()
);
#3256=(
BOUNDED_SURFACE()
B_SPLINE_SURFACE(3,2,((#241209,#241210,#241211),(#241212,#241213,#241214),
(#241215,#241216,#241217),(#241218,#241219,#241220),(#241221,#241222,#241223),
(#241224,#241225,#241226)),.UNSPECIFIED.,.F.,.F.,.F.)
B_SPLINE_SURFACE_WITH_KNOTS((4,2,4),(3,3),(0.,0.000256592814262154,0.000513185628524309),
(0.,1.),.UNSPECIFIED.)
GEOMETRIC_REPRESENTATION_ITEM()
RATIONAL_B_SPLINE_SURFACE(((1.,0.708712527163678,1.),(1.,0.753780902613434,
1.),(1.,0.794538995769399,1.),(1.,0.855070770330911,1.),(1.,0.875018427445479,
1.),(1.,0.874619707139399,1.)))
REPRESENTATION_ITEM('')
SURFACE()
);
#3257=(
BOUNDED_SURFACE()
B_SPLINE_SURFACE(3,2,((#241228,#241229,#241230),(#241231,#241232,#241233),
(#241234,#241235,#241236),(#241237,#241238,#241239)),.UNSPECIFIED.,.F.,
 .F.,.F.)
B_SPLINE_SURFACE_WITH_KNOTS((4,4),(3,3),(0.,0.000511815072430392),(0.,1.00105598365858),
 .UNSPECIFIED.)
GEOMETRIC_REPRESENTATION_ITEM()
RATIONAL_B_SPLINE_SURFACE(((1.,0.70679749073377,1.00061923411688),(1.,0.706182062146689,
1.00062053388194),(1.,0.705584062769055,1.00062179683708),(1.,0.705266224770533,
1.00062246810055)))
REPRESENTATION_ITEM('')
SURFACE()
);
#3258=(
BOUNDED_SURFACE()
B_SPLINE_SURFACE(3,2,((#241245,#241246,#241247),(#241248,#241249,#241250),
(#241251,#241252,#241253),(#241254,#241255,#241256),(#241257,#241258,#241259),
(#241260,#241261,#241262)),.UNSPECIFIED.,.F.,.F.,.F.)
B_SPLINE_SURFACE_WITH_KNOTS((4,2,4),(3,3),(-1.76182853028894E-18,0.000257652232350886,
0.000515304464701773),(0.,1.),.UNSPECIFIED.)
GEOMETRIC_REPRESENTATION_ITEM()
RATIONAL_B_SPLINE_SURFACE(((1.,0.87461970713938,1.),(1.,0.874861180430654,
1.),(1.,0.855455725920906,1.),(1.,0.794699358955208,1.),(1.,0.75376897778866,
1.),(1.,0.708712527163654,1.)))
REPRESENTATION_ITEM('')
SURFACE()
);
#3259=(
BOUNDED_SURFACE()
B_SPLINE_SURFACE(3,2,((#241268,#241269,#241270),(#241271,#241272,#241273),
(#241274,#241275,#241276),(#241277,#241278,#241279)),.UNSPECIFIED.,.F.,
 .F.,.F.)
B_SPLINE_SURFACE_WITH_KNOTS((4,4),(3,3),(-7.23704950134074E-18,0.000397394373651904),
(0.,1.),.UNSPECIFIED.)
GEOMETRIC_REPRESENTATION_ITEM()
RATIONAL_B_SPLINE_SURFACE(((1.,0.707106781186554,1.),(1.,0.707752587915903,
1.),(1.,0.708377654540659,1.),(1.,0.70868977088333,1.)))
REPRESENTATION_ITEM('')
SURFACE()
);
#3260=(
BOUNDED_SURFACE()
B_SPLINE_SURFACE(3,2,((#241281,#241282,#241283),(#241284,#241285,#241286),
(#241287,#241288,#241289),(#241290,#241291,#241292)),.UNSPECIFIED.,.F.,
 .F.,.F.)
B_SPLINE_SURFACE_WITH_KNOTS((4,4),(3,3),(-1.35525271560688E-19,0.000511815456479788),
(0.,1.00105873159961),.UNSPECIFIED.)
GEOMETRIC_REPRESENTATION_ITEM()
RATIONAL_B_SPLINE_SURFACE(((1.,0.708394529056427,1.00061746385341),(1.,
0.708058564166958,1.0006181752467),(1.,0.707430835372167,1.00061950443932),
(1.,0.706796685880481,1.00062084722754)))
REPRESENTATION_ITEM('')
SURFACE()
);
#3261=(
BOUNDED_SURFACE()
B_SPLINE_SURFACE(3,2,((#241298,#241299,#241300),(#241301,#241302,#241303),
(#241304,#241305,#241306),(#241307,#241308,#241309)),.UNSPECIFIED.,.F.,
 .F.,.F.)
B_SPLINE_SURFACE_WITH_KNOTS((4,4),(3,3),(-2.46655994240452E-18,0.000397394465448289),
(0.,1.),.UNSPECIFIED.)
GEOMETRIC_REPRESENTATION_ITEM()
RATIONAL_B_SPLINE_SURFACE(((1.,0.705498956110751,1.),(1.,0.705821764811789,
1.),(1.,0.706461952521142,1.),(1.,0.707106781186545,1.)))
REPRESENTATION_ITEM('')
SURFACE()
);
#3262=(
BOUNDED_SURFACE()
B_SPLINE_SURFACE(3,2,((#241315,#241316,#241317),(#241318,#241319,#241320),
(#241321,#241322,#241323),(#241324,#241325,#241326)),.UNSPECIFIED.,.F.,
 .F.,.F.)
B_SPLINE_SURFACE_WITH_KNOTS((4,4),(3,3),(-3.79470760369927E-19,0.000397394410828735),
(0.,1.),.UNSPECIFIED.)
GEOMETRIC_REPRESENTATION_ITEM()
RATIONAL_B_SPLINE_SURFACE(((1.,0.708689770883326,1.),(1.,0.708376440034481,
1.),(1.,0.707750498698415,1.),(1.,0.707106781186545,1.)))
REPRESENTATION_ITEM('')
SURFACE()
);
#3263=(
BOUNDED_SURFACE()
B_SPLINE_SURFACE(3,2,((#241332,#241333,#241334),(#241335,#241336,#241337),
(#241338,#241339,#241340),(#241341,#241342,#241343)),.UNSPECIFIED.,.F.,
 .F.,.F.)
B_SPLINE_SURFACE_WITH_KNOTS((4,4),(3,3),(0.,0.000511815090126178),(0.,1.00105592270117),
 .UNSPECIFIED.)
GEOMETRIC_REPRESENTATION_ITEM()
RATIONAL_B_SPLINE_SURFACE(((1.,0.705266242717812,1.00062243213023),(1.,
0.705584085909414,1.00062176089455),(1.,0.706182089450808,1.00062049800352),
(1.,0.70679750858778,1.00061919833345)))
REPRESENTATION_ITEM('')
SURFACE()
);
#3264=(
BOUNDED_SURFACE()
B_SPLINE_SURFACE(3,2,((#241345,#241346,#241347),(#241348,#241349,#241350),
(#241351,#241352,#241353),(#241354,#241355,#241356)),.UNSPECIFIED.,.F.,
 .F.,.F.)
B_SPLINE_SURFACE_WITH_KNOTS((4,4),(3,3),(-7.77915058758349E-18,0.000397394428086625),
(0.,1.),.UNSPECIFIED.)
GEOMETRIC_REPRESENTATION_ITEM()
RATIONAL_B_SPLINE_SURFACE(((1.,0.707106781186545,1.),(1.,0.706459846759091,
1.),(1.,0.705820510737286,1.),(1.,0.705498956110761,1.)))
REPRESENTATION_ITEM('')
SURFACE()
);
#3265=(
BOUNDED_SURFACE()
B_SPLINE_SURFACE(3,2,((#241362,#241363,#241364),(#241365,#241366,#241367),
(#241368,#241369,#241370),(#241371,#241372,#241373),(#241374,#241375,#241376),
(#241377,#241378,#241379)),.UNSPECIFIED.,.F.,.F.,.F.)
B_SPLINE_SURFACE_WITH_KNOTS((4,2,4),(3,3),(0.,0.000257953807872846,0.000515907615745691),
(0.,1.),.UNSPECIFIED.)
GEOMETRIC_REPRESENTATION_ITEM()
RATIONAL_B_SPLINE_SURFACE(((1.,0.874619707139396,1.),(1.,0.874834349678915,
1.),(1.,0.85468610415791,1.),(1.,0.792476597915036,1.),(1.,0.750887854595192,
1.),(1.,0.705585838031471,1.)))
REPRESENTATION_ITEM('')
SURFACE()
);
#3266=(
BOUNDED_SURFACE()
B_SPLINE_SURFACE(3,2,((#241385,#241386,#241387),(#241388,#241389,#241390),
(#241391,#241392,#241393),(#241394,#241395,#241396)),.UNSPECIFIED.,.F.,
 .F.,.F.)
B_SPLINE_SURFACE_WITH_KNOTS((4,4),(3,3),(-7.80625564189563E-18,0.00051181543769914),
(0.,1.00105881331477),.UNSPECIFIED.)
GEOMETRIC_REPRESENTATION_ITEM()
RATIONAL_B_SPLINE_SURFACE(((1.,0.706796661946661,1.00062089519653),(1.,
0.707430821225544,1.00061955228395),(1.,0.708058545831046,1.00061822299761),
(1.,0.708394505253034,1.00061751156099)))
REPRESENTATION_ITEM('')
SURFACE()
);
#3267=(
BOUNDED_SURFACE()
B_SPLINE_SURFACE(3,2,((#241398,#241399,#241400),(#241401,#241402,#241403),
(#241404,#241405,#241406),(#241407,#241408,#241409),(#241410,#241411,#241412),
(#241413,#241414,#241415)),.UNSPECIFIED.,.F.,.F.,.F.)
B_SPLINE_SURFACE_WITH_KNOTS((4,2,4),(3,3),(-2.71050543121376E-20,0.000256915317531264,
0.000513830635062527),(0.,1.),.UNSPECIFIED.)
GEOMETRIC_REPRESENTATION_ITEM()
RATIONAL_B_SPLINE_SURFACE(((1.,0.705585838031459,1.),(1.,0.750902433542926,
1.),(1.,0.792329530082281,1.),(1.,0.854288401594456,1.),(1.,0.874998031124951,
1.),(1.,0.874619707139397,1.)))
REPRESENTATION_ITEM('')
SURFACE()
);
#3268=(
BOUNDED_SURFACE()
B_SPLINE_SURFACE(3,2,((#241421,#241422,#241423),(#241424,#241425,#241426),
(#241427,#241428,#241429),(#241430,#241431,#241432),(#241433,#241434,#241435),
(#241436,#241437,#241438)),.UNSPECIFIED.,.F.,.F.,.F.)
B_SPLINE_SURFACE_WITH_KNOTS((4,2,4),(3,3),(-1.02999206386123E-17,0.000256592814262153,
0.000513185628524316),(0.,1.),.UNSPECIFIED.)
GEOMETRIC_REPRESENTATION_ITEM()
RATIONAL_B_SPLINE_SURFACE(((1.,0.708712527163656,1.),(1.,0.75378090261397,
1.),(1.,0.794538995768696,1.),(1.,0.855070770331603,1.),(1.,0.875018427444962,
1.),(1.,0.874619707139397,1.)))
REPRESENTATION_ITEM('')
SURFACE()
);
#3269=(
BOUNDED_SURFACE()
B_SPLINE_SURFACE(3,2,((#241440,#241441,#241442),(#241443,#241444,#241445),
(#241446,#241447,#241448),(#241449,#241450,#241451)),.UNSPECIFIED.,.F.,
 .F.,.F.)
B_SPLINE_SURFACE_WITH_KNOTS((4,4),(3,3),(2.71050543121376E-20,0.000511815072430401),
(0.,1.00105598365924),.UNSPECIFIED.)
GEOMETRIC_REPRESENTATION_ITEM()
RATIONAL_B_SPLINE_SURFACE(((1.,0.706797490733581,1.00061923411727),(1.,
0.706182062146486,1.00062053388233),(1.,0.70558406276887,1.00062179683747),
(1.,0.705266224770332,1.00062246810094)))
REPRESENTATION_ITEM('')
SURFACE()
);
#3270=(
BOUNDED_SURFACE()
B_SPLINE_SURFACE(3,2,((#241457,#241458,#241459),(#241460,#241461,#241462),
(#241463,#241464,#241465),(#241466,#241467,#241468),(#241469,#241470,#241471),
(#241472,#241473,#241474)),.UNSPECIFIED.,.F.,.F.,.F.)
B_SPLINE_SURFACE_WITH_KNOTS((4,2,4),(3,3),(-3.48299947910968E-18,0.000257652232350876,
0.000515304464701756),(0.,1.),.UNSPECIFIED.)
GEOMETRIC_REPRESENTATION_ITEM()
RATIONAL_B_SPLINE_SURFACE(((1.,0.874619707139392,1.),(1.,0.874861180430568,
1.),(1.,0.85545572592103,1.),(1.,0.794699358955112,1.),(1.,0.753768977788717,
1.),(1.,0.708712527163672,1.)))
REPRESENTATION_ITEM('')
SURFACE()
);
#3271=(
BOUNDED_SURFACE()
B_SPLINE_SURFACE(3,2,((#241480,#241481,#241482),(#241483,#241484,#241485),
(#241486,#241487,#241488),(#241489,#241490,#241491)),.UNSPECIFIED.,.F.,
 .F.,.F.)
B_SPLINE_SURFACE_WITH_KNOTS((4,4),(3,3),(0.,0.000397394373651928),(0.,1.),
 .UNSPECIFIED.)
GEOMETRIC_REPRESENTATION_ITEM()
RATIONAL_B_SPLINE_SURFACE(((1.,0.707106781186544,1.),(1.,0.707752587915889,
1.),(1.,0.708377654540682,1.),(1.,0.708689770883336,1.)))
REPRESENTATION_ITEM('')
SURFACE()
);
#3272=(
BOUNDED_SURFACE()
B_SPLINE_SURFACE(3,2,((#241493,#241494,#241495),(#241496,#241497,#241498),
(#241499,#241500,#241501),(#241502,#241503,#241504)),.UNSPECIFIED.,.F.,
 .F.,.F.)
B_SPLINE_SURFACE_WITH_KNOTS((4,4),(3,3),(0.,0.000511815456479792),(0.,1.00105873159925),
 .UNSPECIFIED.)
GEOMETRIC_REPRESENTATION_ITEM()
RATIONAL_B_SPLINE_SURFACE(((1.,0.708394529056543,1.0006174638532),(1.,0.708058564167093,
1.00061817524649),(1.,0.707430835372262,1.00061950443911),(1.,0.706796685880581,
1.00062084722733)))
REPRESENTATION_ITEM('')
SURFACE()
);
#3273=(
BOUNDED_SURFACE()
B_SPLINE_SURFACE(3,2,((#241510,#241511,#241512),(#241513,#241514,#241515),
(#241516,#241517,#241518),(#241519,#241520,#241521)),.UNSPECIFIED.,.F.,
 .F.,.F.)
B_SPLINE_SURFACE_WITH_KNOTS((4,4),(3,3),(3.79470760369927E-19,0.00039739446544831),
(0.,1.),.UNSPECIFIED.)
GEOMETRIC_REPRESENTATION_ITEM()
RATIONAL_B_SPLINE_SURFACE(((1.,0.705498956110749,1.),(1.,0.705821764811784,
1.),(1.,0.70646195252114,1.),(1.,0.707106781186547,1.)))
REPRESENTATION_ITEM('')
SURFACE()
);
#3274=(
BOUNDED_SURFACE()
B_SPLINE_SURFACE(3,2,((#241527,#241528,#241529),(#241530,#241531,#241532),
(#241533,#241534,#241535),(#241536,#241537,#241538)),.UNSPECIFIED.,.F.,
 .F.,.F.)
B_SPLINE_SURFACE_WITH_KNOTS((4,4),(3,3),(-4.87890977618477E-19,0.000397394410828753),
(0.,1.),.UNSPECIFIED.)
GEOMETRIC_REPRESENTATION_ITEM()
RATIONAL_B_SPLINE_SURFACE(((1.,0.708689770883332,1.),(1.,0.70837644003451,
1.),(1.,0.70775049869839,1.),(1.,0.707106781186553,1.)))
REPRESENTATION_ITEM('')
SURFACE()
);
#3275=(
BOUNDED_SURFACE()
B_SPLINE_SURFACE(3,2,((#241544,#241545,#241546),(#241547,#241548,#241549),
(#241550,#241551,#241552),(#241553,#241554,#241555)),.UNSPECIFIED.,.F.,
 .F.,.F.)
B_SPLINE_SURFACE_WITH_KNOTS((4,4),(3,3),(-3.22550146314438E-18,0.000511815090126175),
(0.,1.00105592270393),.UNSPECIFIED.)
GEOMETRIC_REPRESENTATION_ITEM()
RATIONAL_B_SPLINE_SURFACE(((1.,0.705266242717003,1.00062243213186),(1.,
0.705584085908612,1.00062176089618),(1.,0.706182089449985,1.00062049800514),
(1.,0.706797508586972,1.00061919833506)))
REPRESENTATION_ITEM('')
SURFACE()
);
#3276=(
BOUNDED_SURFACE()
B_SPLINE_SURFACE(3,2,((#241557,#241558,#241559),(#241560,#241561,#241562),
(#241563,#241564,#241565),(#241566,#241567,#241568)),.UNSPECIFIED.,.F.,
 .F.,.F.)
B_SPLINE_SURFACE_WITH_KNOTS((4,4),(3,3),(0.,0.000397394428086626),(0.,1.),
 .UNSPECIFIED.)
GEOMETRIC_REPRESENTATION_ITEM()
RATIONAL_B_SPLINE_SURFACE(((1.,0.707106781186545,1.),(1.,0.706459846759104,
1.),(1.,0.705820510737273,1.),(1.,0.705498956110752,1.)))
REPRESENTATION_ITEM('')
SURFACE()
);
#3277=(
BOUNDED_SURFACE()
B_SPLINE_SURFACE(3,2,((#241574,#241575,#241576),(#241577,#241578,#241579),
(#241580,#241581,#241582),(#241583,#241584,#241585),(#241586,#241587,#241588),
(#241589,#241590,#241591)),.UNSPECIFIED.,.F.,.F.,.F.)
B_SPLINE_SURFACE_WITH_KNOTS((4,2,4),(3,3),(0.,0.000257953807872851,0.000515907615745702),
(0.,1.),.UNSPECIFIED.)
GEOMETRIC_REPRESENTATION_ITEM()
RATIONAL_B_SPLINE_SURFACE(((1.,0.874619707139392,1.),(1.,0.874834349678881,
1.),(1.,0.85468610415795,1.),(1.,0.792476597914979,1.),(1.,0.750887854595268,
1.),(1.,0.705585838031435,1.)))
REPRESENTATION_ITEM('')
SURFACE()
);
#3278=(
BOUNDED_SURFACE()
B_SPLINE_SURFACE(3,2,((#241597,#241598,#241599),(#241600,#241601,#241602),
(#241603,#241604,#241605),(#241606,#241607,#241608)),.UNSPECIFIED.,.F.,
 .F.,.F.)
B_SPLINE_SURFACE_WITH_KNOTS((4,4),(3,3),(0.,0.000511815437699157),(0.,1.00105881331701),
 .UNSPECIFIED.)
GEOMETRIC_REPRESENTATION_ITEM()
RATIONAL_B_SPLINE_SURFACE(((1.,0.706796661946011,1.00062089519785),(1.,
0.707430821224864,1.00061955228527),(1.,0.708058545830404,1.00061822299893),
(1.,0.708394505252382,1.00061751156231)))
REPRESENTATION_ITEM('')
SURFACE()
);
#3279=(
BOUNDED_SURFACE()
B_SPLINE_SURFACE(3,2,((#241610,#241611,#241612),(#241613,#241614,#241615),
(#241616,#241617,#241618),(#241619,#241620,#241621),(#241622,#241623,#241624),
(#241625,#241626,#241627)),.UNSPECIFIED.,.F.,.F.,.F.)
B_SPLINE_SURFACE_WITH_KNOTS((4,2,4),(3,3),(1.62630325872826E-19,0.000256915317531262,
0.000513830635062524),(0.,1.),.UNSPECIFIED.)
GEOMETRIC_REPRESENTATION_ITEM()
RATIONAL_B_SPLINE_SURFACE(((1.,0.705585838031439,1.),(1.,0.750902433542569,
1.),(1.,0.792329530082738,1.),(1.,0.854288401593987,1.),(1.,0.874998031125295,
1.),(1.,0.8746197071394,1.)))
REPRESENTATION_ITEM('')
SURFACE()
);
#3280=(
BOUNDED_SURFACE()
B_SPLINE_SURFACE(3,2,((#241633,#241634,#241635),(#241636,#241637,#241638),
(#241639,#241640,#241641),(#241642,#241643,#241644),(#241645,#241646,#241647),
(#241648,#241649,#241650)),.UNSPECIFIED.,.F.,.F.,.F.)
B_SPLINE_SURFACE_WITH_KNOTS((4,2,4),(3,3),(-3.03576608295941E-18,0.000256592814262156,
0.000513185628524315),(0.,1.),.UNSPECIFIED.)
GEOMETRIC_REPRESENTATION_ITEM()
RATIONAL_B_SPLINE_SURFACE(((1.,0.708712527163661,1.),(1.,0.753780902613533,
1.),(1.,0.794538995769294,1.),(1.,0.855070770331017,1.),(1.,0.875018427445396,
1.),(1.,0.874619707139393,1.)))
REPRESENTATION_ITEM('')
SURFACE()
);
#3281=(
BOUNDED_SURFACE()
B_SPLINE_SURFACE(3,2,((#241652,#241653,#241654),(#241655,#241656,#241657),
(#241658,#241659,#241660),(#241661,#241662,#241663)),.UNSPECIFIED.,.F.,
 .F.,.F.)
B_SPLINE_SURFACE_WITH_KNOTS((4,4),(3,3),(0.,0.000511815072430393),(0.,1.00105598365816),
 .UNSPECIFIED.)
GEOMETRIC_REPRESENTATION_ITEM()
RATIONAL_B_SPLINE_SURFACE(((1.,0.706797490733887,1.00061923411664),(1.,
0.706182062146832,1.0006205338817),(1.,0.705584062769154,1.00062179683684),
(1.,0.705266224770657,1.0006224681003)))
REPRESENTATION_ITEM('')
SURFACE()
);
#3282=(
BOUNDED_SURFACE()
B_SPLINE_SURFACE(3,2,((#241669,#241670,#241671),(#241672,#241673,#241674),
(#241675,#241676,#241677),(#241678,#241679,#241680),(#241681,#241682,#241683),
(#241684,#241685,#241686)),.UNSPECIFIED.,.F.,.F.,.F.)
B_SPLINE_SURFACE_WITH_KNOTS((4,2,4),(3,3),(5.28548559086683E-19,0.000257652232350874,
0.000515304464701748),(0.,1.),.UNSPECIFIED.)
GEOMETRIC_REPRESENTATION_ITEM()
RATIONAL_B_SPLINE_SURFACE(((1.,0.874619707139394,1.),(1.,0.8748611804306,
1.),(1.,0.855455725921013,1.),(1.,0.794699358955116,1.),(1.,0.753768977788727,
1.),(1.,0.708712527163692,1.)))
REPRESENTATION_ITEM('')
SURFACE()
);
#3283=(
BOUNDED_SURFACE()
B_SPLINE_SURFACE(3,2,((#241692,#241693,#241694),(#241695,#241696,#241697),
(#241698,#241699,#241700),(#241701,#241702,#241703)),.UNSPECIFIED.,.F.,
 .F.,.F.)
B_SPLINE_SURFACE_WITH_KNOTS((4,4),(3,3),(0.,0.000397394373651919),(0.,1.),
 .UNSPECIFIED.)
GEOMETRIC_REPRESENTATION_ITEM()
RATIONAL_B_SPLINE_SURFACE(((1.,0.70710678118655,1.),(1.,0.707752587915875,
1.),(1.,0.708377654540735,1.),(1.,0.708689770883314,1.)))
REPRESENTATION_ITEM('')
SURFACE()
);
#3284=(
BOUNDED_SURFACE()
B_SPLINE_SURFACE(3,2,((#241705,#241706,#241707),(#241708,#241709,#241710),
(#241711,#241712,#241713),(#241714,#241715,#241716)),.UNSPECIFIED.,.F.,
 .F.,.F.)
B_SPLINE_SURFACE_WITH_KNOTS((4,4),(3,3),(0.,0.000511815456479785),(0.,1.00105873160019),
 .UNSPECIFIED.)
GEOMETRIC_REPRESENTATION_ITEM()
RATIONAL_B_SPLINE_SURFACE(((1.,0.708394529056267,1.00061746385375),(1.,
0.708058564166825,1.00061817524704),(1.,0.707430835372014,1.00061950443966),
(1.,0.706796685880295,1.00062084722788)))
REPRESENTATION_ITEM('')
SURFACE()
);
#3285=(
BOUNDED_SURFACE()
B_SPLINE_SURFACE(3,2,((#241722,#241723,#241724),(#241725,#241726,#241727),
(#241728,#241729,#241730),(#241731,#241732,#241733)),.UNSPECIFIED.,.F.,
 .F.,.F.)
B_SPLINE_SURFACE_WITH_KNOTS((4,4),(3,3),(4.87890977618477E-19,0.000397394465448305),
(0.,1.),.UNSPECIFIED.)
GEOMETRIC_REPRESENTATION_ITEM()
RATIONAL_B_SPLINE_SURFACE(((1.,0.705498956110739,1.),(1.,0.705821764811805,
1.),(1.,0.706461952521113,1.),(1.,0.707106781186559,1.)))
REPRESENTATION_ITEM('')
SURFACE()
);
#3286=(
BOUNDED_SURFACE()
B_SPLINE_SURFACE(3,2,((#241739,#241740,#241741),(#241742,#241743,#241744),
(#241745,#241746,#241747),(#241748,#241749,#241750)),.UNSPECIFIED.,.F.,
 .F.,.F.)
B_SPLINE_SURFACE_WITH_KNOTS((4,4),(3,3),(-5.96311194867027E-19,0.000397394410828722),
(0.,1.),.UNSPECIFIED.)
GEOMETRIC_REPRESENTATION_ITEM()
RATIONAL_B_SPLINE_SURFACE(((1.,0.708689770883324,1.),(1.,0.708376440034489,
1.),(1.,0.707750498698425,1.),(1.,0.707106781186535,1.)))
REPRESENTATION_ITEM('')
SURFACE()
);
#3287=(
BOUNDED_SURFACE()
B_SPLINE_SURFACE(3,2,((#241756,#241757,#241758),(#241759,#241760,#241761),
(#241762,#241763,#241764),(#241765,#241766,#241767)),.UNSPECIFIED.,.F.,
 .F.,.F.)
B_SPLINE_SURFACE_WITH_KNOTS((4,4),(3,3),(0.,0.000511815090126176),(0.,1.00105592270271),
 .UNSPECIFIED.)
GEOMETRIC_REPRESENTATION_ITEM()
RATIONAL_B_SPLINE_SURFACE(((1.,0.705266242717332,1.00062243213114),(1.,
0.705584085908974,1.00062176089545),(1.,0.706182089450373,1.00062049800442),
(1.,0.706797508587321,1.00061919833435)))
REPRESENTATION_ITEM('')
SURFACE()
);
#3288=(
BOUNDED_SURFACE()
B_SPLINE_SURFACE(3,2,((#241769,#241770,#241771),(#241772,#241773,#241774),
(#241775,#241776,#241777),(#241778,#241779,#241780)),.UNSPECIFIED.,.F.,
 .F.,.F.)
B_SPLINE_SURFACE_WITH_KNOTS((4,4),(3,3),(-8.13151629364128E-20,0.000397394428086617),
(0.,1.),.UNSPECIFIED.)
GEOMETRIC_REPRESENTATION_ITEM()
RATIONAL_B_SPLINE_SURFACE(((1.,0.707106781186563,1.),(1.,0.706459846759093,
1.),(1.,0.705820510737283,1.),(1.,0.705498956110757,1.)))
REPRESENTATION_ITEM('')
SURFACE()
);
#3289=(
BOUNDED_SURFACE()
B_SPLINE_SURFACE(3,2,((#241786,#241787,#241788),(#241789,#241790,#241791),
(#241792,#241793,#241794),(#241795,#241796,#241797),(#241798,#241799,#241800),
(#241801,#241802,#241803)),.UNSPECIFIED.,.F.,.F.,.F.)
B_SPLINE_SURFACE_WITH_KNOTS((4,2,4),(3,3),(0.,0.000257953807872855,0.00051590761574571),
(0.,1.),.UNSPECIFIED.)
GEOMETRIC_REPRESENTATION_ITEM()
RATIONAL_B_SPLINE_SURFACE(((1.,0.874619707139394,1.),(1.,0.874834349678904,
1.),(1.,0.854686104157903,1.),(1.,0.792476597915017,1.),(1.,0.750887854595213,
1.),(1.,0.705585838031453,1.)))
REPRESENTATION_ITEM('')
SURFACE()
);
#3290=(
BOUNDED_SURFACE()
B_SPLINE_SURFACE(3,2,((#241809,#241810,#241811),(#241812,#241813,#241814),
(#241815,#241816,#241817),(#241818,#241819,#241820)),.UNSPECIFIED.,.F.,
 .F.,.F.)
B_SPLINE_SURFACE_WITH_KNOTS((4,4),(3,3),(0.,0.000511815437699146),(0.,1.00105881331748),
 .UNSPECIFIED.)
GEOMETRIC_REPRESENTATION_ITEM()
RATIONAL_B_SPLINE_SURFACE(((1.,0.706796661945865,1.00062089519812),(1.,
0.707430821224745,1.00061955228554),(1.,0.708058545830274,1.0006182229992),
(1.,0.708394505252235,1.00061751156258)))
REPRESENTATION_ITEM('')
SURFACE()
);
#3291=(
BOUNDED_SURFACE()
B_SPLINE_SURFACE(3,2,((#241822,#241823,#241824),(#241825,#241826,#241827),
(#241828,#241829,#241830),(#241831,#241832,#241833),(#241834,#241835,#241836),
(#241837,#241838,#241839)),.UNSPECIFIED.,.F.,.F.,.F.)
B_SPLINE_SURFACE_WITH_KNOTS((4,2,4),(3,3),(3.52365706057789E-19,0.00025691531753126,
0.00051383063506252),(0.,1.),.UNSPECIFIED.)
GEOMETRIC_REPRESENTATION_ITEM()
RATIONAL_B_SPLINE_SURFACE(((1.,0.705585838031451,1.),(1.,0.750902433542401,
1.),(1.,0.79232953008298,1.),(1.,0.854288401593769,1.),(1.,0.874998031125475,
1.),(1.,0.874619707139399,1.)))
REPRESENTATION_ITEM('')
SURFACE()
);
#3292=(
BOUNDED_SURFACE()
B_SPLINE_SURFACE(3,2,((#241845,#241846,#241847),(#241848,#241849,#241850),
(#241851,#241852,#241853),(#241854,#241855,#241856),(#241857,#241858,#241859),
(#241860,#241861,#241862)),.UNSPECIFIED.,.F.,.F.,.F.)
B_SPLINE_SURFACE_WITH_KNOTS((4,2,4),(3,3),(-4.30970363562988E-18,0.000256592814262152,
0.000513185628524307),(0.,1.),.UNSPECIFIED.)
GEOMETRIC_REPRESENTATION_ITEM()
RATIONAL_B_SPLINE_SURFACE(((1.,0.708712527163664,1.),(1.,0.753780902613362,
1.),(1.,0.794538995769504,1.),(1.,0.855070770330797,1.),(1.,0.875018427445572,
1.),(1.,0.874619707139393,1.)))
REPRESENTATION_ITEM('')
SURFACE()
);
#3293=(
BOUNDED_SURFACE()
B_SPLINE_SURFACE(3,2,((#241864,#241865,#241866),(#241867,#241868,#241869),
(#241870,#241871,#241872),(#241873,#241874,#241875)),.UNSPECIFIED.,.F.,
 .F.,.F.)
B_SPLINE_SURFACE_WITH_KNOTS((4,4),(3,3),(5.6920614055489E-19,0.000511815072430397),
(0.,1.00105598365966),.UNSPECIFIED.)
GEOMETRIC_REPRESENTATION_ITEM()
RATIONAL_B_SPLINE_SURFACE(((1.,0.706797490733448,1.00061923411751),(1.,
0.70618206214638,1.00062053388258),(1.,0.705584062768717,1.00062179683772),
(1.,0.705266224770207,1.00062246810119)))
REPRESENTATION_ITEM('')
SURFACE()
);
#3294=(
BOUNDED_SURFACE()
B_SPLINE_SURFACE(3,2,((#241881,#241882,#241883),(#241884,#241885,#241886),
(#241887,#241888,#241889),(#241890,#241891,#241892),(#241893,#241894,#241895),
(#241896,#241897,#241898)),.UNSPECIFIED.,.F.,.F.,.F.)
B_SPLINE_SURFACE_WITH_KNOTS((4,2,4),(3,3),(-3.19839640883224E-18,0.000257652232350882,
0.000515304464701768),(0.,1.),.UNSPECIFIED.)
GEOMETRIC_REPRESENTATION_ITEM()
RATIONAL_B_SPLINE_SURFACE(((1.,0.874619707139399,1.),(1.,0.874861180430683,
1.),(1.,0.855455725920874,1.),(1.,0.794699358955272,1.),(1.,0.753768977788643,
1.),(1.,0.708712527163664,1.)))
REPRESENTATION_ITEM('')
SURFACE()
);
#3295=(
BOUNDED_SURFACE()
B_SPLINE_SURFACE(3,2,((#241904,#241905,#241906),(#241907,#241908,#241909),
(#241910,#241911,#241912),(#241913,#241914,#241915)),.UNSPECIFIED.,.F.,
 .F.,.F.)
B_SPLINE_SURFACE_WITH_KNOTS((4,4),(3,3),(0.,0.000397394373651913),(0.,1.),
 .UNSPECIFIED.)
GEOMETRIC_REPRESENTATION_ITEM()
RATIONAL_B_SPLINE_SURFACE(((1.,0.70710678118654,1.),(1.,0.707752587915903,
1.),(1.,0.708377654540674,1.),(1.,0.708689770883327,1.)))
REPRESENTATION_ITEM('')
SURFACE()
);
#3296=(
BOUNDED_SURFACE()
B_SPLINE_SURFACE(3,2,((#241917,#241918,#241919),(#241920,#241921,#241922),
(#241923,#241924,#241925),(#241926,#241927,#241928)),.UNSPECIFIED.,.F.,
 .F.,.F.)
B_SPLINE_SURFACE_WITH_KNOTS((4,4),(3,3),(0.,0.000511815456479788),(0.,1.00105873159895),
 .UNSPECIFIED.)
GEOMETRIC_REPRESENTATION_ITEM()
RATIONAL_B_SPLINE_SURFACE(((1.,0.708394529056624,1.00061746385303),(1.,
0.708058564167179,1.00061817524632),(1.,0.70743083537233,1.00061950443894),
(1.,0.706796685880683,1.00062084722715)))
REPRESENTATION_ITEM('')
SURFACE()
);
#3297=(
BOUNDED_SURFACE()
B_SPLINE_SURFACE(3,2,((#241934,#241935,#241936),(#241937,#241938,#241939),
(#241940,#241941,#241942),(#241943,#241944,#241945)),.UNSPECIFIED.,.F.,
 .F.,.F.)
B_SPLINE_SURFACE_WITH_KNOTS((4,4),(3,3),(-1.43656787854329E-18,0.000397394465448297),
(0.,1.),.UNSPECIFIED.)
GEOMETRIC_REPRESENTATION_ITEM()
RATIONAL_B_SPLINE_SURFACE(((1.,0.70549895611075,1.),(1.,0.705821764811781,
1.),(1.,0.706461952521137,1.),(1.,0.70710678118655,1.)))
REPRESENTATION_ITEM('')
SURFACE()
);
#3298=(
BOUNDED_SURFACE()
B_SPLINE_SURFACE(3,2,((#241951,#241952,#241953),(#241954,#241955,#241956),
(#241957,#241958,#241959),(#241960,#241961,#241962)),.UNSPECIFIED.,.F.,
 .F.,.F.)
B_SPLINE_SURFACE_WITH_KNOTS((4,4),(3,3),(0.,0.000397394410828738),(0.,1.),
 .UNSPECIFIED.)
GEOMETRIC_REPRESENTATION_ITEM()
RATIONAL_B_SPLINE_SURFACE(((1.,0.708689770883318,1.),(1.,0.708376440034509,
1.),(1.,0.707750498698355,1.),(1.,0.707106781186568,1.)))
REPRESENTATION_ITEM('')
SURFACE()
);
#3299=(
BOUNDED_SURFACE()
B_SPLINE_SURFACE(3,2,((#241968,#241969,#241970),(#241971,#241972,#241973),
(#241974,#241975,#241976),(#241977,#241978,#241979)),.UNSPECIFIED.,.F.,
 .F.,.F.)
B_SPLINE_SURFACE_WITH_KNOTS((4,4),(3,3),(0.,0.00051181509012617),(0.,1.00105592270631),
 .UNSPECIFIED.)
GEOMETRIC_REPRESENTATION_ITEM()
RATIONAL_B_SPLINE_SURFACE(((1.,0.705266242716285,1.00062243213326),(1.,
0.705584085907913,1.00062176089758),(1.,0.706182089449311,1.00062049800654),
(1.,0.706797508586264,1.00061919833646)))
REPRESENTATION_ITEM('')
SURFACE()
);
#3300=(
BOUNDED_SURFACE()
B_SPLINE_SURFACE(3,2,((#241981,#241982,#241983),(#241984,#241985,#241986),
(#241987,#241988,#241989),(#241990,#241991,#241992)),.UNSPECIFIED.,.F.,
 .F.,.F.)
B_SPLINE_SURFACE_WITH_KNOTS((4,4),(3,3),(0.,0.000397394428086615),(0.,1.),
 .UNSPECIFIED.)
GEOMETRIC_REPRESENTATION_ITEM()
RATIONAL_B_SPLINE_SURFACE(((1.,0.707106781186545,1.),(1.,0.706459846759086,
1.),(1.,0.70582051073728,1.),(1.,0.70549895611076,1.)))
REPRESENTATION_ITEM('')
SURFACE()
);
#3301=(
BOUNDED_SURFACE()
B_SPLINE_SURFACE(3,2,((#241998,#241999,#242000),(#242001,#242002,#242003),
(#242004,#242005,#242006),(#242007,#242008,#242009),(#242010,#242011,#242012),
(#242013,#242014,#242015)),.UNSPECIFIED.,.F.,.F.,.F.)
B_SPLINE_SURFACE_WITH_KNOTS((4,2,4),(3,3),(0.,0.000257953807872855,0.000515907615745711),
(0.,1.),.UNSPECIFIED.)
GEOMETRIC_REPRESENTATION_ITEM()
RATIONAL_B_SPLINE_SURFACE(((1.,0.87461970713939,1.),(1.,0.874834349678975,
1.),(1.,0.854686104157832,1.),(1.,0.7924765979151,1.),(1.,0.750887854595135,
1.),(1.,0.705585838031471,1.)))
REPRESENTATION_ITEM('')
SURFACE()
);
#3302=(
BOUNDED_SURFACE()
B_SPLINE_SURFACE(3,2,((#242021,#242022,#242023),(#242024,#242025,#242026),
(#242027,#242028,#242029),(#242030,#242031,#242032)),.UNSPECIFIED.,.F.,
 .F.,.F.)
B_SPLINE_SURFACE_WITH_KNOTS((4,4),(3,3),(-6.26126754610379E-18,0.000511815437699142),
(0.,1.00105881331519),.UNSPECIFIED.)
GEOMETRIC_REPRESENTATION_ITEM()
RATIONAL_B_SPLINE_SURFACE(((1.,0.70679666194653,1.00062089519678),(1.,0.707430821225431,
1.0006195522842),(1.,0.708058545830899,1.00061822299786),(1.,0.708394505252917,
1.00061751156124)))
REPRESENTATION_ITEM('')
SURFACE()
);
#3303=(
BOUNDED_SURFACE()
B_SPLINE_SURFACE(3,2,((#242034,#242035,#242036),(#242037,#242038,#242039),
(#242040,#242041,#242042),(#242043,#242044,#242045),(#242046,#242047,#242048),
(#242049,#242050,#242051)),.UNSPECIFIED.,.F.,.F.,.F.)
B_SPLINE_SURFACE_WITH_KNOTS((4,2,4),(3,3),(0.,0.000256915317531255,0.00051383063506251),
(0.,1.),.UNSPECIFIED.)
GEOMETRIC_REPRESENTATION_ITEM()
RATIONAL_B_SPLINE_SURFACE(((1.,0.705585838031438,1.),(1.,0.750902433542754,
1.),(1.,0.792329530082518,1.),(1.,0.854288401594195,1.),(1.,0.874998031125136,
1.),(1.,0.874619707139401,1.)))
REPRESENTATION_ITEM('')
SURFACE()
);
#3304=(
BOUNDED_SURFACE()
B_SPLINE_SURFACE(3,2,((#242057,#242058,#242059),(#242060,#242061,#242062),
(#242063,#242064,#242065),(#242066,#242067,#242068),(#242069,#242070,#242071),
(#242072,#242073,#242074)),.UNSPECIFIED.,.F.,.F.,.F.)
B_SPLINE_SURFACE_WITH_KNOTS((4,2,4),(3,3),(0.,0.000256592814262162,0.000513185628524325),
(0.,1.),.UNSPECIFIED.)
GEOMETRIC_REPRESENTATION_ITEM()
RATIONAL_B_SPLINE_SURFACE(((1.,0.708712527163663,1.),(1.,0.753780902613412,
1.),(1.,0.794538995769447,1.),(1.,0.855070770330856,1.),(1.,0.875018427445525,
1.),(1.,0.87461970713939,1.)))
REPRESENTATION_ITEM('')
SURFACE()
);
#3305=(
BOUNDED_SURFACE()
B_SPLINE_SURFACE(3,2,((#242076,#242077,#242078),(#242079,#242080,#242081),
(#242082,#242083,#242084),(#242085,#242086,#242087)),.UNSPECIFIED.,.F.,
 .F.,.F.)
B_SPLINE_SURFACE_WITH_KNOTS((4,4),(3,3),(-2.71050543121376E-20,0.000511815072430413),
(0.,1.00105598365856),.UNSPECIFIED.)
GEOMETRIC_REPRESENTATION_ITEM()
RATIONAL_B_SPLINE_SURFACE(((1.,0.70679749073378,1.00061923411687),(1.,0.706182062146706,
1.00062053388193),(1.,0.70558406276906,1.00062179683707),(1.,0.705266224770537,
1.00062246810054)))
REPRESENTATION_ITEM('')
SURFACE()
);
#3306=(
BOUNDED_SURFACE()
B_SPLINE_SURFACE(3,2,((#242093,#242094,#242095),(#242096,#242097,#242098),
(#242099,#242100,#242101),(#242102,#242103,#242104),(#242105,#242106,#242107),
(#242108,#242109,#242110)),.UNSPECIFIED.,.F.,.F.,.F.)
B_SPLINE_SURFACE_WITH_KNOTS((4,2,4),(3,3),(-8.13151629364128E-20,0.000257652232350874,
0.000515304464701749),(0.,1.),.UNSPECIFIED.)
GEOMETRIC_REPRESENTATION_ITEM()
RATIONAL_B_SPLINE_SURFACE(((1.,0.874619707139396,1.),(1.,0.874861180430513,
1.),(1.,0.855455725921131,1.),(1.,0.794699358954991,1.),(1.,0.753768977788884,
1.),(1.,0.708712527163653,1.)))
REPRESENTATION_ITEM('')
SURFACE()
);
#3307=(
BOUNDED_SURFACE()
B_SPLINE_SURFACE(3,2,((#242116,#242117,#242118),(#242119,#242120,#242121),
(#242122,#242123,#242124),(#242125,#242126,#242127)),.UNSPECIFIED.,.F.,
 .F.,.F.)
B_SPLINE_SURFACE_WITH_KNOTS((4,4),(3,3),(-1.04083408558608E-17,0.000397394373651904),
(0.,1.),.UNSPECIFIED.)
GEOMETRIC_REPRESENTATION_ITEM()
RATIONAL_B_SPLINE_SURFACE(((1.,0.70710678118655,1.),(1.,0.707752587915888,
1.),(1.,0.708377654540711,1.),(1.,0.708689770883332,1.)))
REPRESENTATION_ITEM('')
SURFACE()
);
#3308=(
BOUNDED_SURFACE()
B_SPLINE_SURFACE(3,2,((#242129,#242130,#242131),(#242132,#242133,#242134),
(#242135,#242136,#242137),(#242138,#242139,#242140)),.UNSPECIFIED.,.F.,
 .F.,.F.)
B_SPLINE_SURFACE_WITH_KNOTS((4,4),(3,3),(-3.6049722235143E-18,0.000511815456479789),
(0.,1.00105873159758),.UNSPECIFIED.)
GEOMETRIC_REPRESENTATION_ITEM()
RATIONAL_B_SPLINE_SURFACE(((1.,0.708394529057025,1.00061746385223),(1.,
0.708058564167564,1.00061817524552),(1.,0.70743083537276,1.00061950443814),
(1.,0.706796685881074,1.00062084722635)))
REPRESENTATION_ITEM('')
SURFACE()
);
#3309=(
BOUNDED_SURFACE()
B_SPLINE_SURFACE(3,2,((#242146,#242147,#242148),(#242149,#242150,#242151),
(#242152,#242153,#242154),(#242155,#242156,#242157)),.UNSPECIFIED.,.F.,
 .F.,.F.)
B_SPLINE_SURFACE_WITH_KNOTS((4,4),(3,3),(0.,0.000397394465448303),(0.,1.),
 .UNSPECIFIED.)
GEOMETRIC_REPRESENTATION_ITEM()
RATIONAL_B_SPLINE_SURFACE(((1.,0.705498956110737,1.),(1.,0.70582176481177,
1.),(1.,0.70646195252114,1.),(1.,0.70710678118655,1.)))
REPRESENTATION_ITEM('')
SURFACE()
);
#3310=(
BOUNDED_SURFACE()
B_SPLINE_SURFACE(3,2,((#242163,#242164,#242165),(#242166,#242167,#242168),
(#242169,#242170,#242171),(#242172,#242173,#242174)),.UNSPECIFIED.,.F.,
 .F.,.F.)
B_SPLINE_SURFACE_WITH_KNOTS((4,4),(3,3),(0.,0.000397394410828738),(0.,1.),
 .UNSPECIFIED.)
GEOMETRIC_REPRESENTATION_ITEM()
RATIONAL_B_SPLINE_SURFACE(((1.,0.708689770883326,1.),(1.,0.708376440034507,
1.),(1.,0.707750498698402,1.),(1.,0.707106781186546,1.)))
REPRESENTATION_ITEM('')
SURFACE()
);
#3311=(
BOUNDED_SURFACE()
B_SPLINE_SURFACE(3,2,((#242180,#242181,#242182),(#242183,#242184,#242185),
(#242186,#242187,#242188),(#242189,#242190,#242191)),.UNSPECIFIED.,.F.,
 .F.,.F.)
B_SPLINE_SURFACE_WITH_KNOTS((4,4),(3,3),(-1.62630325872826E-18,0.000511815090126177),
(0.,1.0010559227041),.UNSPECIFIED.)
GEOMETRIC_REPRESENTATION_ITEM()
RATIONAL_B_SPLINE_SURFACE(((1.,0.705266242716925,1.00062243213196),(1.,
0.705584085908534,1.00062176089627),(1.,0.706182089449937,1.00062049800524),
(1.,0.706797508586938,1.00061919833516)))
REPRESENTATION_ITEM('')
SURFACE()
);
#3312=(
BOUNDED_SURFACE()
B_SPLINE_SURFACE(3,2,((#242193,#242194,#242195),(#242196,#242197,#242198),
(#242199,#242200,#242201),(#242202,#242203,#242204)),.UNSPECIFIED.,.F.,
 .F.,.F.)
B_SPLINE_SURFACE_WITH_KNOTS((4,4),(3,3),(0.,0.000397394428086624),(0.,1.),
 .UNSPECIFIED.)
GEOMETRIC_REPRESENTATION_ITEM()
RATIONAL_B_SPLINE_SURFACE(((1.,0.707106781186533,1.),(1.,0.706459846759113,
1.),(1.,0.705820510737269,1.),(1.,0.705498956110716,1.)))
REPRESENTATION_ITEM('')
SURFACE()
);
#3313=(
BOUNDED_SURFACE()
B_SPLINE_SURFACE(3,2,((#242210,#242211,#242212),(#242213,#242214,#242215),
(#242216,#242217,#242218),(#242219,#242220,#242221),(#242222,#242223,#242224),
(#242225,#242226,#242227)),.UNSPECIFIED.,.F.,.F.,.F.)
B_SPLINE_SURFACE_WITH_KNOTS((4,2,4),(3,3),(0.,0.000257953807872849,0.000515907615745699),
(0.,1.),.UNSPECIFIED.)
GEOMETRIC_REPRESENTATION_ITEM()
RATIONAL_B_SPLINE_SURFACE(((1.,0.874619707139391,1.),(1.,0.874834349679018,
1.),(1.,0.854686104157772,1.),(1.,0.792476597915156,1.),(1.,0.750887854595126,
1.),(1.,0.705585838031422,1.)))
REPRESENTATION_ITEM('')
SURFACE()
);
#3314=(
BOUNDED_SURFACE()
B_SPLINE_SURFACE(3,2,((#242233,#242234,#242235),(#242236,#242237,#242238),
(#242239,#242240,#242241),(#242242,#242243,#242244)),.UNSPECIFIED.,.F.,
 .F.,.F.)
B_SPLINE_SURFACE_WITH_KNOTS((4,4),(3,3),(0.,0.000511815437699142),(0.,1.00105881331444),
 .UNSPECIFIED.)
GEOMETRIC_REPRESENTATION_ITEM()
RATIONAL_B_SPLINE_SURFACE(((1.,0.706796661946758,1.00062089519634),(1.,
0.707430821225624,1.00061955228376),(1.,0.70805854583117,1.00061822299742),
(1.,0.708394505253132,1.0006175115608)))
REPRESENTATION_ITEM('')
SURFACE()
);
#3315=(
BOUNDED_SURFACE()
B_SPLINE_SURFACE(3,2,((#242246,#242247,#242248),(#242249,#242250,#242251),
(#242252,#242253,#242254),(#242255,#242256,#242257),(#242258,#242259,#242260),
(#242261,#242262,#242263)),.UNSPECIFIED.,.F.,.F.,.F.)
B_SPLINE_SURFACE_WITH_KNOTS((4,2,4),(3,3),(2.71050543121376E-20,0.00025691531753127,
0.000513830635062539),(0.,1.),.UNSPECIFIED.)
GEOMETRIC_REPRESENTATION_ITEM()
RATIONAL_B_SPLINE_SURFACE(((1.,0.705585838031442,1.),(1.,0.750902433543051,
1.),(1.,0.792329530082094,1.),(1.,0.854288401594649,1.),(1.,0.8749980311248,
1.),(1.,0.874619707139398,1.)))
REPRESENTATION_ITEM('')
SURFACE()
);
#3316=(
BOUNDED_SURFACE()
B_SPLINE_SURFACE(3,2,((#242269,#242270,#242271),(#242272,#242273,#242274),
(#242275,#242276,#242277),(#242278,#242279,#242280),(#242281,#242282,#242283),
(#242284,#242285,#242286)),.UNSPECIFIED.,.F.,.F.,.F.)
B_SPLINE_SURFACE_WITH_KNOTS((4,2,4),(3,3),(-1.11401773222886E-17,0.000256592814262152,
0.000513185628524315),(0.,1.),.UNSPECIFIED.)
GEOMETRIC_REPRESENTATION_ITEM()
RATIONAL_B_SPLINE_SURFACE(((1.,0.708712527163676,1.),(1.,0.753780902613421,
1.),(1.,0.794538995769422,1.),(1.,0.855070770330898,1.),(1.,0.875018427445499,
1.),(1.,0.874619707139395,1.)))
REPRESENTATION_ITEM('')
SURFACE()
);
#3317=(
BOUNDED_SURFACE()
B_SPLINE_SURFACE(3,2,((#242288,#242289,#242290),(#242291,#242292,#242293),
(#242294,#242295,#242296),(#242297,#242298,#242299)),.UNSPECIFIED.,.F.,
 .F.,.F.)
B_SPLINE_SURFACE_WITH_KNOTS((4,4),(3,3),(-1.62630325872826E-19,0.000511815072430405),
(0.,1.00105598365847),.UNSPECIFIED.)
GEOMETRIC_REPRESENTATION_ITEM()
RATIONAL_B_SPLINE_SURFACE(((1.,0.706797490733806,1.00061923411681),(1.,
0.706182062146721,1.00062053388188),(1.,0.705584062769095,1.00062179683702),
(1.,0.705266224770575,1.00062246810048)))
REPRESENTATION_ITEM('')
SURFACE()
);
#3318=(
BOUNDED_SURFACE()
B_SPLINE_SURFACE(3,2,((#242305,#242306,#242307),(#242308,#242309,#242310),
(#242311,#242312,#242313),(#242314,#242315,#242316),(#242317,#242318,#242319),
(#242320,#242321,#242322)),.UNSPECIFIED.,.F.,.F.,.F.)
B_SPLINE_SURFACE_WITH_KNOTS((4,2,4),(3,3),(0.,0.000257652232350882,0.000515304464701764),
(0.,1.),.UNSPECIFIED.)
GEOMETRIC_REPRESENTATION_ITEM()
RATIONAL_B_SPLINE_SURFACE(((1.,0.874619707139392,1.),(1.,0.874861180430873,
1.),(1.,0.855455725920652,1.),(1.,0.79469935895548,1.),(1.,0.753768977788454,
1.),(1.,0.708712527163685,1.)))
REPRESENTATION_ITEM('')
SURFACE()
);
#3319=(
BOUNDED_SURFACE()
B_SPLINE_SURFACE(3,2,((#242328,#242329,#242330),(#242331,#242332,#242333),
(#242334,#242335,#242336),(#242337,#242338,#242339)),.UNSPECIFIED.,.F.,
 .F.,.F.)
B_SPLINE_SURFACE_WITH_KNOTS((4,4),(3,3),(-7.31836466427715E-19,0.000397394373651924),
(0.,1.),.UNSPECIFIED.)
GEOMETRIC_REPRESENTATION_ITEM()
RATIONAL_B_SPLINE_SURFACE(((1.,0.707106781186549,1.),(1.,0.707752587915856,
1.),(1.,0.708377654540692,1.),(1.,0.708689770883325,1.)))
REPRESENTATION_ITEM('')
SURFACE()
);
#3320=(
BOUNDED_SURFACE()
B_SPLINE_SURFACE(3,2,((#242341,#242342,#242343),(#242344,#242345,#242346),
(#242347,#242348,#242349),(#242350,#242351,#242352)),.UNSPECIFIED.,.F.,
 .F.,.F.)
B_SPLINE_SURFACE_WITH_KNOTS((4,4),(3,3),(0.,0.000511815456479794),(0.,1.00105873159879),
 .UNSPECIFIED.)
GEOMETRIC_REPRESENTATION_ITEM()
RATIONAL_B_SPLINE_SURFACE(((1.,0.708394529056662,1.00061746385294),(1.,
0.70805856416723,1.00061817524622),(1.,0.707430835372382,1.00061950443885),
(1.,0.70679668588072,1.00062084722706)))
REPRESENTATION_ITEM('')
SURFACE()
);
#3321=(
BOUNDED_SURFACE()
B_SPLINE_SURFACE(3,2,((#242358,#242359,#242360),(#242361,#242362,#242363),
(#242364,#242365,#242366),(#242367,#242368,#242369)),.UNSPECIFIED.,.F.,
 .F.,.F.)
B_SPLINE_SURFACE_WITH_KNOTS((4,4),(3,3),(-4.06575814682064E-18,0.0003973944654483),
(0.,1.),.UNSPECIFIED.)
GEOMETRIC_REPRESENTATION_ITEM()
RATIONAL_B_SPLINE_SURFACE(((1.,0.705498956110753,1.),(1.,0.705821764811809,
1.),(1.,0.706461952521118,1.),(1.,0.707106781186563,1.)))
REPRESENTATION_ITEM('')
SURFACE()
);
#3322=(
BOUNDED_SURFACE()
B_SPLINE_SURFACE(3,2,((#242375,#242376,#242377),(#242378,#242379,#242380),
(#242381,#242382,#242383),(#242384,#242385,#242386)),.UNSPECIFIED.,.F.,
 .F.,.F.)
B_SPLINE_SURFACE_WITH_KNOTS((4,4),(3,3),(0.,0.000397394410828732),(0.,1.),
 .UNSPECIFIED.)
GEOMETRIC_REPRESENTATION_ITEM()
RATIONAL_B_SPLINE_SURFACE(((1.,0.708689770883298,1.),(1.,0.708376440034519,
1.),(1.,0.707750498698387,1.),(1.,0.707106781186546,1.)))
REPRESENTATION_ITEM('')
SURFACE()
);
#3323=(
BOUNDED_SURFACE()
B_SPLINE_SURFACE(3,2,((#242392,#242393,#242394),(#242395,#242396,#242397),
(#242398,#242399,#242400),(#242401,#242402,#242403)),.UNSPECIFIED.,.F.,
 .F.,.F.)
B_SPLINE_SURFACE_WITH_KNOTS((4,4),(3,3),(-3.22550146314438E-18,0.000511815090126175),
(0.,1.00105592270367),.UNSPECIFIED.)
GEOMETRIC_REPRESENTATION_ITEM()
RATIONAL_B_SPLINE_SURFACE(((1.,0.705266242717061,1.00062243213171),(1.,
0.705584085908694,1.00062176089602),(1.,0.706182089450076,1.00062049800499),
(1.,0.70679750858705,1.00061919833491)))
REPRESENTATION_ITEM('')
SURFACE()
);
#3324=(
BOUNDED_SURFACE()
B_SPLINE_SURFACE(3,2,((#242405,#242406,#242407),(#242408,#242409,#242410),
(#242411,#242412,#242413),(#242414,#242415,#242416)),.UNSPECIFIED.,.F.,
 .F.,.F.)
B_SPLINE_SURFACE_WITH_KNOTS((4,4),(3,3),(-4.66206934168767E-18,0.000397394428086629),
(0.,1.),.UNSPECIFIED.)
GEOMETRIC_REPRESENTATION_ITEM()
RATIONAL_B_SPLINE_SURFACE(((1.,0.707106781186546,1.),(1.,0.706459846759078,
1.),(1.,0.705820510737287,1.),(1.,0.705498956110751,1.)))
REPRESENTATION_ITEM('')
SURFACE()
);
#3325=(
BOUNDED_SURFACE()
B_SPLINE_SURFACE(3,2,((#242422,#242423,#242424),(#242425,#242426,#242427),
(#242428,#242429,#242430),(#242431,#242432,#242433),(#242434,#242435,#242436),
(#242437,#242438,#242439)),.UNSPECIFIED.,.F.,.F.,.F.)
B_SPLINE_SURFACE_WITH_KNOTS((4,2,4),(3,3),(0.,0.000257953807872843,0.000515907615745686),
(0.,1.),.UNSPECIFIED.)
GEOMETRIC_REPRESENTATION_ITEM()
RATIONAL_B_SPLINE_SURFACE(((1.,0.874619707139389,1.),(1.,0.874834349678801,
1.),(1.,0.854686104158044,1.),(1.,0.792476597914911,1.),(1.,0.750887854595285,
1.),(1.,0.705585838031442,1.)))
REPRESENTATION_ITEM('')
SURFACE()
);
#3326=(
BOUNDED_SURFACE()
B_SPLINE_SURFACE(3,2,((#242445,#242446,#242447),(#242448,#242449,#242450),
(#242451,#242452,#242453),(#242454,#242455,#242456)),.UNSPECIFIED.,.F.,
 .F.,.F.)
B_SPLINE_SURFACE_WITH_KNOTS((4,4),(3,3),(-1.03812358015487E-17,0.00051181543769915),
(0.,1.00105881331573),.UNSPECIFIED.)
GEOMETRIC_REPRESENTATION_ITEM()
RATIONAL_B_SPLINE_SURFACE(((1.,0.70679666194638,1.00062089519709),(1.,0.707430821225288,
1.00061955228452),(1.,0.708058545830734,1.00061822299818),(1.,0.708394505252756,
1.00061751156156)))
REPRESENTATION_ITEM('')
SURFACE()
);
#3327=(
BOUNDED_SURFACE()
B_SPLINE_SURFACE(3,2,((#242458,#242459,#242460),(#242461,#242462,#242463),
(#242464,#242465,#242466),(#242467,#242468,#242469),(#242470,#242471,#242472),
(#242473,#242474,#242475)),.UNSPECIFIED.,.F.,.F.,.F.)
B_SPLINE_SURFACE_WITH_KNOTS((4,2,4),(3,3),(0.,0.00025691531753126,0.000513830635062521),
(0.,1.),.UNSPECIFIED.)
GEOMETRIC_REPRESENTATION_ITEM()
RATIONAL_B_SPLINE_SURFACE(((1.,0.705585838031422,1.),(1.,0.750902433542275,
1.),(1.,0.792329530083122,1.),(1.,0.854288401593586,1.),(1.,0.874998031125599,
1.),(1.,0.874619707139391,1.)))
REPRESENTATION_ITEM('')
SURFACE()
);
#3328=(
BOUNDED_SURFACE()
B_SPLINE_SURFACE(3,2,((#242481,#242482,#242483),(#242484,#242485,#242486),
(#242487,#242488,#242489),(#242490,#242491,#242492),(#242493,#242494,#242495),
(#242496,#242497,#242498)),.UNSPECIFIED.,.F.,.F.,.F.)
B_SPLINE_SURFACE_WITH_KNOTS((4,2,4),(3,3),(-2.16840434497101E-18,0.000256592814262155,
0.000513185628524311),(0.,1.),.UNSPECIFIED.)
GEOMETRIC_REPRESENTATION_ITEM()
RATIONAL_B_SPLINE_SURFACE(((1.,0.708712527163659,1.),(1.,0.753780902613598,
1.),(1.,0.794538995769182,1.),(1.,0.855070770331133,1.),(1.,0.875018427445305,
1.),(1.,0.874619707139401,1.)))
REPRESENTATION_ITEM('')
SURFACE()
);
#3329=(
BOUNDED_SURFACE()
B_SPLINE_SURFACE(3,2,((#242500,#242501,#242502),(#242503,#242504,#242505),
(#242506,#242507,#242508),(#242509,#242510,#242511)),.UNSPECIFIED.,.F.,
 .F.,.F.)
B_SPLINE_SURFACE_WITH_KNOTS((4,4),(3,3),(0.,0.000511815072430405),(0.,1.00105598365859),
 .UNSPECIFIED.)
GEOMETRIC_REPRESENTATION_ITEM()
RATIONAL_B_SPLINE_SURFACE(((1.,0.70679749073377,1.00061923411689),(1.,0.706182062146715,
1.00062053388195),(1.,0.705584062769003,1.00062179683709),(1.,0.705266224770533,
1.00062246810055)))
REPRESENTATION_ITEM('')
SURFACE()
);
#3330=(
BOUNDED_SURFACE()
B_SPLINE_SURFACE(3,2,((#242517,#242518,#242519),(#242520,#242521,#242522),
(#242523,#242524,#242525),(#242526,#242527,#242528),(#242529,#242530,#242531),
(#242532,#242533,#242534)),.UNSPECIFIED.,.F.,.F.,.F.)
B_SPLINE_SURFACE_WITH_KNOTS((4,2,4),(3,3),(4.47233396150271E-19,0.000257652232350877,
0.000515304464701754),(0.,1.),.UNSPECIFIED.)
GEOMETRIC_REPRESENTATION_ITEM()
RATIONAL_B_SPLINE_SURFACE(((1.,0.874619707139385,1.),(1.,0.874861180431084,
1.),(1.,0.855455725920359,1.),(1.,0.794699358955758,1.),(1.,0.753768977788267,
1.),(1.,0.708712527163679,1.)))
REPRESENTATION_ITEM('')
SURFACE()
);
#3331=(
BOUNDED_SURFACE()
B_SPLINE_SURFACE(3,2,((#242540,#242541,#242542),(#242543,#242544,#242545),
(#242546,#242547,#242548),(#242549,#242550,#242551)),.UNSPECIFIED.,.F.,
 .F.,.F.)
B_SPLINE_SURFACE_WITH_KNOTS((4,4),(3,3),(0.,0.000397394373651925),(0.,1.),
 .UNSPECIFIED.)
GEOMETRIC_REPRESENTATION_ITEM()
RATIONAL_B_SPLINE_SURFACE(((1.,0.707106781186536,1.),(1.,0.707752587915914,
1.),(1.,0.708377654540683,1.),(1.,0.708689770883341,1.)))
REPRESENTATION_ITEM('')
SURFACE()
);
#3332=(
BOUNDED_SURFACE()
B_SPLINE_SURFACE(3,2,((#242553,#242554,#242555),(#242556,#242557,#242558),
(#242559,#242560,#242561),(#242562,#242563,#242564)),.UNSPECIFIED.,.F.,
 .F.,.F.)
B_SPLINE_SURFACE_WITH_KNOTS((4,4),(3,3),(0.,0.000511815456479785),(0.,1.00105873159772),
 .UNSPECIFIED.)
GEOMETRIC_REPRESENTATION_ITEM()
RATIONAL_B_SPLINE_SURFACE(((1.,0.708394529056973,1.00061746385231),(1.,
0.708058564167544,1.0006181752456),(1.,0.707430835372716,1.00061950443822),
(1.,0.706796685881033,1.00062084722643)))
REPRESENTATION_ITEM('')
SURFACE()
);
#3333=(
BOUNDED_SURFACE()
B_SPLINE_SURFACE(3,2,((#242570,#242571,#242572),(#242573,#242574,#242575),
(#242576,#242577,#242578),(#242579,#242580,#242581)),.UNSPECIFIED.,.F.,
 .F.,.F.)
B_SPLINE_SURFACE_WITH_KNOTS((4,4),(3,3),(0.,0.0003973944654483),(0.,1.),
 .UNSPECIFIED.)
GEOMETRIC_REPRESENTATION_ITEM()
RATIONAL_B_SPLINE_SURFACE(((1.,0.705498956110768,1.),(1.,0.705821764811725,
1.),(1.,0.706461952521167,1.),(1.,0.707106781186562,1.)))
REPRESENTATION_ITEM('')
SURFACE()
);
#3334=(
BOUNDED_SURFACE()
B_SPLINE_SURFACE(3,2,((#242587,#242588,#242589),(#242590,#242591,#242592),
(#242593,#242594,#242595),(#242596,#242597,#242598)),.UNSPECIFIED.,.F.,
 .F.,.F.)
B_SPLINE_SURFACE_WITH_KNOTS((4,4),(3,3),(0.,0.000397394410828727),(0.,1.),
 .UNSPECIFIED.)
GEOMETRIC_REPRESENTATION_ITEM()
RATIONAL_B_SPLINE_SURFACE(((1.,0.708689770883342,1.),(1.,0.708376440034501,
1.),(1.,0.707750498698418,1.),(1.,0.707106781186535,1.)))
REPRESENTATION_ITEM('')
SURFACE()
);
#3335=(
BOUNDED_SURFACE()
B_SPLINE_SURFACE(3,2,((#242604,#242605,#242606),(#242607,#242608,#242609),
(#242610,#242611,#242612),(#242613,#242614,#242615)),.UNSPECIFIED.,.F.,
 .F.,.F.)
B_SPLINE_SURFACE_WITH_KNOTS((4,4),(3,3),(0.,0.000511815090126171),(0.,1.00105592270294),
 .UNSPECIFIED.)
GEOMETRIC_REPRESENTATION_ITEM()
RATIONAL_B_SPLINE_SURFACE(((1.,0.705266242717261,1.00062243213128),(1.,
0.70558408590891,1.00062176089559),(1.,0.706182089450261,1.00062049800456),
(1.,0.706797508587264,1.00061919833448)))
REPRESENTATION_ITEM('')
SURFACE()
);
#3336=(
BOUNDED_SURFACE()
B_SPLINE_SURFACE(3,2,((#242617,#242618,#242619),(#242620,#242621,#242622),
(#242623,#242624,#242625),(#242626,#242627,#242628)),.UNSPECIFIED.,.F.,
 .F.,.F.)
B_SPLINE_SURFACE_WITH_KNOTS((4,4),(3,3),(-5.09575021068187E-18,0.000397394428086616),
(0.,1.),.UNSPECIFIED.)
GEOMETRIC_REPRESENTATION_ITEM()
RATIONAL_B_SPLINE_SURFACE(((1.,0.707106781186535,1.),(1.,0.706459846759122,
1.),(1.,0.705820510737254,1.),(1.,0.705498956110735,1.)))
REPRESENTATION_ITEM('')
SURFACE()
);
#3337=(
BOUNDED_SURFACE()
B_SPLINE_SURFACE(3,2,((#242634,#242635,#242636),(#242637,#242638,#242639),
(#242640,#242641,#242642),(#242643,#242644,#242645),(#242646,#242647,#242648),
(#242649,#242650,#242651)),.UNSPECIFIED.,.F.,.F.,.F.)
B_SPLINE_SURFACE_WITH_KNOTS((4,2,4),(3,3),(0.,0.000257953807872844,0.000515907615745688),
(0.,1.),.UNSPECIFIED.)
GEOMETRIC_REPRESENTATION_ITEM()
RATIONAL_B_SPLINE_SURFACE(((1.,0.874619707139395,1.),(1.,0.87483434967913,
1.),(1.,0.854686104157619,1.),(1.,0.792476597915322,1.),(1.,0.750887854595009,
1.),(1.,0.705585838031439,1.)))
REPRESENTATION_ITEM('')
SURFACE()
);
#3338=(
BOUNDED_SURFACE()
B_SPLINE_SURFACE(3,2,((#242657,#242658,#242659),(#242660,#242661,#242662),
(#242663,#242664,#242665),(#242666,#242667,#242668)),.UNSPECIFIED.,.F.,
 .F.,.F.)
B_SPLINE_SURFACE_WITH_KNOTS((4,4),(3,3),(0.,0.000511815437699143),(0.,1.001058813316),
 .UNSPECIFIED.)
GEOMETRIC_REPRESENTATION_ITEM()
RATIONAL_B_SPLINE_SURFACE(((1.,0.706796661946313,1.00062089519725),(1.,
0.707430821225155,1.00061955228467),(1.,0.708058545830717,1.00061822299833),
(1.,0.708394505252681,1.00061751156171)))
REPRESENTATION_ITEM('')
SURFACE()
);
#3339=(
BOUNDED_SURFACE()
B_SPLINE_SURFACE(3,2,((#242670,#242671,#242672),(#242673,#242674,#242675),
(#242676,#242677,#242678),(#242679,#242680,#242681),(#242682,#242683,#242684),
(#242685,#242686,#242687)),.UNSPECIFIED.,.F.,.F.,.F.)
B_SPLINE_SURFACE_WITH_KNOTS((4,2,4),(3,3),(-6.50521303491303E-18,0.000256915317531246,
0.000513830635062499),(0.,1.),.UNSPECIFIED.)
GEOMETRIC_REPRESENTATION_ITEM()
RATIONAL_B_SPLINE_SURFACE(((1.,0.70558583803145,1.),(1.,0.750902433541874,
1.),(1.,0.792329530083662,1.),(1.,0.854288401593093,1.),(1.,0.874998031125971,
1.),(1.,0.874619707139399,1.)))
REPRESENTATION_ITEM('')
SURFACE()
);
#3340=(
BOUNDED_SURFACE()
B_SPLINE_SURFACE(3,2,((#242693,#242694,#242695),(#242696,#242697,#242698),
(#242699,#242700,#242701),(#242702,#242703,#242704),(#242705,#242706,#242707),
(#242708,#242709,#242710)),.UNSPECIFIED.,.F.,.F.,.F.)
B_SPLINE_SURFACE_WITH_KNOTS((4,2,4),(3,3),(-9.2970336290632E-18,0.000256592814262158,
0.000513185628524325),(0.,1.),.UNSPECIFIED.)
GEOMETRIC_REPRESENTATION_ITEM()
RATIONAL_B_SPLINE_SURFACE(((1.,0.70871252716368,1.),(1.,0.753780902613021,
1.),(1.,0.79453899576993,1.),(1.,0.855070770330385,1.),(1.,0.875018427445874,
1.),(1.,0.874619707139391,1.)))
REPRESENTATION_ITEM('')
SURFACE()
);
#3341=(
BOUNDED_SURFACE()
B_SPLINE_SURFACE(3,2,((#242712,#242713,#242714),(#242715,#242716,#242717),
(#242718,#242719,#242720),(#242721,#242722,#242723)),.UNSPECIFIED.,.F.,
 .F.,.F.)
B_SPLINE_SURFACE_WITH_KNOTS((4,4),(3,3),(-9.83913471530595E-18,0.0005118150724304),
(0.,1.00105598365781),.UNSPECIFIED.)
GEOMETRIC_REPRESENTATION_ITEM()
RATIONAL_B_SPLINE_SURFACE(((1.,0.706797490733999,1.00061923411643),(1.,
0.706182062146929,1.00062053388149),(1.,0.705584062769251,1.00062179683663),
(1.,0.705266224770772,1.00062246810009)))
REPRESENTATION_ITEM('')
SURFACE()
);
#3342=(
BOUNDED_SURFACE()
B_SPLINE_SURFACE(3,2,((#242729,#242730,#242731),(#242732,#242733,#242734),
(#242735,#242736,#242737),(#242738,#242739,#242740),(#242741,#242742,#242743),
(#242744,#242745,#242746)),.UNSPECIFIED.,.F.,.F.,.F.)
B_SPLINE_SURFACE_WITH_KNOTS((4,2,4),(3,3),(0.,0.000257652232350873,0.000515304464701747),
(0.,1.),.UNSPECIFIED.)
GEOMETRIC_REPRESENTATION_ITEM()
RATIONAL_B_SPLINE_SURFACE(((1.,0.874619707139395,1.),(1.,0.874861180430483,
1.),(1.,0.855455725921158,1.),(1.,0.794699358955009,1.),(1.,0.753768977788842,
1.),(1.,0.708712527163647,1.)))
REPRESENTATION_ITEM('')
SURFACE()
);
#3343=(
BOUNDED_SURFACE()
B_SPLINE_SURFACE(3,2,((#242752,#242753,#242754),(#242755,#242756,#242757),
(#242758,#242759,#242760),(#242761,#242762,#242763)),.UNSPECIFIED.,.F.,
 .F.,.F.)
B_SPLINE_SURFACE_WITH_KNOTS((4,4),(3,3),(-5.66495635123676E-18,0.000397394373651917),
(0.,1.),.UNSPECIFIED.)
GEOMETRIC_REPRESENTATION_ITEM()
RATIONAL_B_SPLINE_SURFACE(((1.,0.707106781186537,1.),(1.,0.707752587915902,
1.),(1.,0.70837765454068,1.),(1.,0.708689770883311,1.)))
REPRESENTATION_ITEM('')
SURFACE()
);
#3344=(
BOUNDED_SURFACE()
B_SPLINE_SURFACE(3,2,((#242765,#242766,#242767),(#242768,#242769,#242770),
(#242771,#242772,#242773),(#242774,#242775,#242776)),.UNSPECIFIED.,.F.,
 .F.,.F.)
B_SPLINE_SURFACE_WITH_KNOTS((4,4),(3,3),(0.,0.000511815456479785),(0.,1.00105873160024),
 .UNSPECIFIED.)
GEOMETRIC_REPRESENTATION_ITEM()
RATIONAL_B_SPLINE_SURFACE(((1.,0.708394529056231,1.00061746385378),(1.,
0.708058564166822,1.00061817524707),(1.,0.707430835371943,1.00061950443969),
(1.,0.706796685880296,1.00062084722791)))
REPRESENTATION_ITEM('')
SURFACE()
);
#3345=(
BOUNDED_SURFACE()
B_SPLINE_SURFACE(3,2,((#242782,#242783,#242784),(#242785,#242786,#242787),
(#242788,#242789,#242790),(#242791,#242792,#242793)),.UNSPECIFIED.,.F.,
 .F.,.F.)
B_SPLINE_SURFACE_WITH_KNOTS((4,4),(3,3),(0.,0.000397394465448315),(0.,1.),
 .UNSPECIFIED.)
GEOMETRIC_REPRESENTATION_ITEM()
RATIONAL_B_SPLINE_SURFACE(((1.,0.705498956110737,1.),(1.,0.705821764811864,
1.),(1.,0.706461952521089,1.),(1.,0.707106781186549,1.)))
REPRESENTATION_ITEM('')
SURFACE()
);
#3346=(
BOUNDED_SURFACE()
B_SPLINE_SURFACE(3,2,((#242799,#242800,#242801),(#242802,#242803,#242804),
(#242805,#242806,#242807),(#242808,#242809,#242810)),.UNSPECIFIED.,.F.,
 .F.,.F.)
B_SPLINE_SURFACE_WITH_KNOTS((4,4),(3,3),(0.,0.000397394410828729),(0.,1.),
 .UNSPECIFIED.)
GEOMETRIC_REPRESENTATION_ITEM()
RATIONAL_B_SPLINE_SURFACE(((1.,0.708689770883334,1.),(1.,0.708376440034477,
1.),(1.,0.70775049869843,1.),(1.,0.707106781186535,1.)))
REPRESENTATION_ITEM('')
SURFACE()
);
#3347=(
BOUNDED_SURFACE()
B_SPLINE_SURFACE(3,2,((#242816,#242817,#242818),(#242819,#242820,#242821),
(#242822,#242823,#242824),(#242825,#242826,#242827)),.UNSPECIFIED.,.F.,
 .F.,.F.)
B_SPLINE_SURFACE_WITH_KNOTS((4,4),(3,3),(0.,0.000511815090126169),(0.,1.00105592270366),
 .UNSPECIFIED.)
GEOMETRIC_REPRESENTATION_ITEM()
RATIONAL_B_SPLINE_SURFACE(((1.,0.705266242717034,1.0006224321317),(1.,0.705584085908732,
1.00062176089601),(1.,0.706182089450059,1.00062049800498),(1.,0.706797508587054,
1.0006191983349)))
REPRESENTATION_ITEM('')
SURFACE()
);
#3348=(
BOUNDED_SURFACE()
B_SPLINE_SURFACE(3,2,((#242829,#242830,#242831),(#242832,#242833,#242834),
(#242835,#242836,#242837),(#242838,#242839,#242840)),.UNSPECIFIED.,.F.,
 .F.,.F.)
B_SPLINE_SURFACE_WITH_KNOTS((4,4),(3,3),(-7.77915058758349E-18,0.00039739442808661),
(0.,1.),.UNSPECIFIED.)
GEOMETRIC_REPRESENTATION_ITEM()
RATIONAL_B_SPLINE_SURFACE(((1.,0.707106781186537,1.),(1.,0.706459846759104,
1.),(1.,0.70582051073728,1.),(1.,0.705498956110748,1.)))
REPRESENTATION_ITEM('')
SURFACE()
);
#3349=(
BOUNDED_SURFACE()
B_SPLINE_SURFACE(3,2,((#242846,#242847,#242848),(#242849,#242850,#242851),
(#242852,#242853,#242854),(#242855,#242856,#242857),(#242858,#242859,#242860),
(#242861,#242862,#242863)),.UNSPECIFIED.,.F.,.F.,.F.)
B_SPLINE_SURFACE_WITH_KNOTS((4,2,4),(3,3),(0.,0.000257953807872845,0.000515907615745691),
(0.,1.),.UNSPECIFIED.)
GEOMETRIC_REPRESENTATION_ITEM()
RATIONAL_B_SPLINE_SURFACE(((1.,0.874619707139393,1.),(1.,0.874834349679444,
1.),(1.,0.854686104157216,1.),(1.,0.792476597915716,1.),(1.,0.75088785459471,
1.),(1.,0.705585838031437,1.)))
REPRESENTATION_ITEM('')
SURFACE()
);
#3350=(
BOUNDED_SURFACE()
B_SPLINE_SURFACE(3,2,((#242869,#242870,#242871),(#242872,#242873,#242874),
(#242875,#242876,#242877),(#242878,#242879,#242880)),.UNSPECIFIED.,.F.,
 .F.,.F.)
B_SPLINE_SURFACE_WITH_KNOTS((4,4),(3,3),(-7.83336069620777E-18,0.000511815437699145),
(0.,1.00105881331516),.UNSPECIFIED.)
GEOMETRIC_REPRESENTATION_ITEM()
RATIONAL_B_SPLINE_SURFACE(((1.,0.706796661946547,1.00062089519676),(1.,
0.70743082122544,1.00061955228419),(1.,0.708058545830902,1.00061822299785),
(1.,0.708394505252928,1.00061751156123)))
REPRESENTATION_ITEM('')
SURFACE()
);
#3351=(
BOUNDED_SURFACE()
B_SPLINE_SURFACE(3,2,((#242882,#242883,#242884),(#242885,#242886,#242887),
(#242888,#242889,#242890),(#242891,#242892,#242893),(#242894,#242895,#242896),
(#242897,#242898,#242899)),.UNSPECIFIED.,.F.,.F.,.F.)
B_SPLINE_SURFACE_WITH_KNOTS((4,2,4),(3,3),(0.,0.000256915317531267,0.000513830635062534),
(0.,1.),.UNSPECIFIED.)
GEOMETRIC_REPRESENTATION_ITEM()
RATIONAL_B_SPLINE_SURFACE(((1.,0.705585838031457,1.),(1.,0.750902433542621,
1.),(1.,0.792329530082714,1.),(1.,0.854288401594055,1.),(1.,0.874998031125253,
1.),(1.,0.874619707139418,1.)))
REPRESENTATION_ITEM('')
SURFACE()
);
#3352=(
BOUNDED_SURFACE()
B_SPLINE_SURFACE(3,2,((#242905,#242906,#242907),(#242908,#242909,#242910),
(#242911,#242912,#242913),(#242914,#242915,#242916),(#242917,#242918,#242919),
(#242920,#242921,#242922)),.UNSPECIFIED.,.F.,.F.,.F.)
B_SPLINE_SURFACE_WITH_KNOTS((4,2,4),(3,3),(2.90024081139872E-18,0.000256592814262166,
0.000513185628524329),(0.,1.),.UNSPECIFIED.)
GEOMETRIC_REPRESENTATION_ITEM()
RATIONAL_B_SPLINE_SURFACE(((1.,0.708712527163643,1.),(1.,0.753780902613616,
1.),(1.,0.794538995769188,1.),(1.,0.855070770331141,1.),(1.,0.875018427445299,
1.),(1.,0.874619707139395,1.)))
REPRESENTATION_ITEM('')
SURFACE()
);
#3353=(
BOUNDED_SURFACE()
B_SPLINE_SURFACE(3,2,((#242924,#242925,#242926),(#242927,#242928,#242929),
(#242930,#242931,#242932),(#242933,#242934,#242935)),.UNSPECIFIED.,.F.,
 .F.,.F.)
B_SPLINE_SURFACE_WITH_KNOTS((4,4),(3,3),(0.,0.0005118150724304),(0.,1.00105598366053),
 .UNSPECIFIED.)
GEOMETRIC_REPRESENTATION_ITEM()
RATIONAL_B_SPLINE_SURFACE(((1.,0.706797490733202,1.00061923411802),(1.,
0.706182062146141,1.00062053388309),(1.,0.705584062768469,1.00062179683823),
(1.,0.705266224769957,1.0006224681017)))
REPRESENTATION_ITEM('')
SURFACE()
);
#3354=(
BOUNDED_SURFACE()
B_SPLINE_SURFACE(3,2,((#242941,#242942,#242943),(#242944,#242945,#242946),
(#242947,#242948,#242949),(#242950,#242951,#242952),(#242953,#242954,#242955),
(#242956,#242957,#242958)),.UNSPECIFIED.,.F.,.F.,.F.)
B_SPLINE_SURFACE_WITH_KNOTS((4,2,4),(3,3),(2.84603070277445E-18,0.000257652232350877,
0.000515304464701752),(0.,1.),.UNSPECIFIED.)
GEOMETRIC_REPRESENTATION_ITEM()
RATIONAL_B_SPLINE_SURFACE(((1.,0.87461970713938,1.),(1.,0.874861180430414,
1.),(1.,0.855455725921217,1.),(1.,0.794699358954895,1.),(1.,0.753768977788904,
1.),(1.,0.708712527163652,1.)))
REPRESENTATION_ITEM('')
SURFACE()
);
#3355=(
BOUNDED_SURFACE()
B_SPLINE_SURFACE(3,2,((#242964,#242965,#242966),(#242967,#242968,#242969),
(#242970,#242971,#242972),(#242973,#242974,#242975)),.UNSPECIFIED.,.F.,
 .F.,.F.)
B_SPLINE_SURFACE_WITH_KNOTS((4,4),(3,3),(-5.42101086242752E-20,0.000397394373651934),
(0.,1.),.UNSPECIFIED.)
GEOMETRIC_REPRESENTATION_ITEM()
RATIONAL_B_SPLINE_SURFACE(((1.,0.70710678118654,1.),(1.,0.707752587915909,
1.),(1.,0.708377654540641,1.),(1.,0.708689770883352,1.)))
REPRESENTATION_ITEM('')
SURFACE()
);
#3356=(
BOUNDED_SURFACE()
B_SPLINE_SURFACE(3,2,((#242977,#242978,#242979),(#242980,#242981,#242982),
(#242983,#242984,#242985),(#242986,#242987,#242988)),.UNSPECIFIED.,.F.,
 .F.,.F.)
B_SPLINE_SURFACE_WITH_KNOTS((4,4),(3,3),(-2.00577401909818E-18,0.000511815456479787),
(0.,1.00105873160032),.UNSPECIFIED.)
GEOMETRIC_REPRESENTATION_ITEM()
RATIONAL_B_SPLINE_SURFACE(((1.,0.708394529056217,1.00061746385383),(1.,
0.708058564166775,1.00061817524712),(1.,0.707430835371947,1.00061950443974),
(1.,0.70679668588027,1.00062084722796)))
REPRESENTATION_ITEM('')
SURFACE()
);
#3357=(
BOUNDED_SURFACE()
B_SPLINE_SURFACE(3,2,((#242994,#242995,#242996),(#242997,#242998,#242999),
(#243000,#243001,#243002),(#243003,#243004,#243005)),.UNSPECIFIED.,.F.,
 .F.,.F.)
B_SPLINE_SURFACE_WITH_KNOTS((4,4),(3,3),(0.,0.000397394465448307),(0.,1.),
 .UNSPECIFIED.)
GEOMETRIC_REPRESENTATION_ITEM()
RATIONAL_B_SPLINE_SURFACE(((1.,0.705498956110759,1.),(1.,0.705821764811783,
1.),(1.,0.706461952521134,1.),(1.,0.70710678118655,1.)))
REPRESENTATION_ITEM('')
SURFACE()
);
#3358=(
BOUNDED_SURFACE()
B_SPLINE_SURFACE(3,2,((#243011,#243012,#243013),(#243014,#243015,#243016),
(#243017,#243018,#243019),(#243020,#243021,#243022)),.UNSPECIFIED.,.F.,
 .F.,.F.)
B_SPLINE_SURFACE_WITH_KNOTS((4,4),(3,3),(0.,0.000397394410828732),(0.,1.),
 .UNSPECIFIED.)
GEOMETRIC_REPRESENTATION_ITEM()
RATIONAL_B_SPLINE_SURFACE(((1.,0.708689770883336,1.),(1.,0.708376440034493,
1.),(1.,0.707750498698416,1.),(1.,0.707106781186546,1.)))
REPRESENTATION_ITEM('')
SURFACE()
);
#3359=(
BOUNDED_SURFACE()
B_SPLINE_SURFACE(3,2,((#243028,#243029,#243030),(#243031,#243032,#243033),
(#243034,#243035,#243036),(#243037,#243038,#243039)),.UNSPECIFIED.,.F.,
 .F.,.F.)
B_SPLINE_SURFACE_WITH_KNOTS((4,4),(3,3),(0.,0.000511815090126173),(0.,1.00105592270393),
 .UNSPECIFIED.)
GEOMETRIC_REPRESENTATION_ITEM()
RATIONAL_B_SPLINE_SURFACE(((1.,0.705266242716976,1.00062243213186),(1.,
0.7055840859086,1.00062176089618),(1.,0.706182089450005,1.00062049800514),
(1.,0.706797508586974,1.00061919833506)))
REPRESENTATION_ITEM('')
SURFACE()
);
#3360=(
BOUNDED_SURFACE()
B_SPLINE_SURFACE(3,2,((#243041,#243042,#243043),(#243044,#243045,#243046),
(#243047,#243048,#243049),(#243050,#243051,#243052)),.UNSPECIFIED.,.F.,
 .F.,.F.)
B_SPLINE_SURFACE_WITH_KNOTS((4,4),(3,3),(-1.51246203061728E-17,0.000397394428086612),
(0.,1.),.UNSPECIFIED.)
GEOMETRIC_REPRESENTATION_ITEM()
RATIONAL_B_SPLINE_SURFACE(((1.,0.707106781186538,1.),(1.,0.706459846759089,
1.),(1.,0.705820510737279,1.),(1.,0.70549895611075,1.)))
REPRESENTATION_ITEM('')
SURFACE()
);
#3361=(
BOUNDED_SURFACE()
B_SPLINE_SURFACE(3,2,((#243058,#243059,#243060),(#243061,#243062,#243063),
(#243064,#243065,#243066),(#243067,#243068,#243069),(#243070,#243071,#243072),
(#243073,#243074,#243075)),.UNSPECIFIED.,.F.,.F.,.F.)
B_SPLINE_SURFACE_WITH_KNOTS((4,2,4),(3,3),(0.,0.000257953807872853,0.000515907615745706),
(0.,1.),.UNSPECIFIED.)
GEOMETRIC_REPRESENTATION_ITEM()
RATIONAL_B_SPLINE_SURFACE(((1.,0.874619707139391,1.),(1.,0.874834349679083,
1.),(1.,0.85468610415769,1.),(1.,0.79247659791523,1.),(1.,0.750887854595076,
1.),(1.,0.705585838031431,1.)))
REPRESENTATION_ITEM('')
SURFACE()
);
#3362=(
BOUNDED_SURFACE()
B_SPLINE_SURFACE(3,2,((#243081,#243082,#243083),(#243084,#243085,#243086),
(#243087,#243088,#243089),(#243090,#243091,#243092)),.UNSPECIFIED.,.F.,
 .F.,.F.)
B_SPLINE_SURFACE_WITH_KNOTS((4,4),(3,3),(-8.13151629364128E-20,0.00051181543769915),
(0.,1.00105881331554),.UNSPECIFIED.)
GEOMETRIC_REPRESENTATION_ITEM()
RATIONAL_B_SPLINE_SURFACE(((1.,0.706796661946445,1.00062089519698),(1.,
0.707430821225321,1.0006195522844),(1.,0.708058545830804,1.00061822299806),
(1.,0.708394505252852,1.00061751156144)))
REPRESENTATION_ITEM('')
SURFACE()
);
#3363=(
BOUNDED_SURFACE()
B_SPLINE_SURFACE(3,2,((#243094,#243095,#243096),(#243097,#243098,#243099),
(#243100,#243101,#243102),(#243103,#243104,#243105),(#243106,#243107,#243108),
(#243109,#243110,#243111)),.UNSPECIFIED.,.F.,.F.,.F.)
B_SPLINE_SURFACE_WITH_KNOTS((4,2,4),(3,3),(-1.05709711817337E-18,0.000256915317531255,
0.000513830635062511),(0.,1.),.UNSPECIFIED.)
GEOMETRIC_REPRESENTATION_ITEM()
RATIONAL_B_SPLINE_SURFACE(((1.,0.705585838031441,1.),(1.,0.750902433542587,
1.),(1.,0.792329530082719,1.),(1.,0.854288401594003,1.),(1.,0.874998031125281,
1.),(1.,0.874619707139393,1.)))
REPRESENTATION_ITEM('')
SURFACE()
);
#3364=(
BOUNDED_SURFACE()
B_SPLINE_SURFACE(3,2,((#243117,#243118,#243119),(#243120,#243121,#243122),
(#243123,#243124,#243125),(#243126,#243127,#243128),(#243129,#243130,#243131),
(#243132,#243133,#243134)),.UNSPECIFIED.,.F.,.F.,.F.)
B_SPLINE_SURFACE_WITH_KNOTS((4,2,4),(3,3),(0.,0.000256592814262157,0.000513185628524314),
(0.,1.),.UNSPECIFIED.)
GEOMETRIC_REPRESENTATION_ITEM()
RATIONAL_B_SPLINE_SURFACE(((1.,0.708712527163663,1.),(1.,0.753780902613579,
1.),(1.,0.794538995769226,1.),(1.,0.855070770331072,1.),(1.,0.875018427445355,
1.),(1.,0.874619707139399,1.)))
REPRESENTATION_ITEM('')
SURFACE()
);
#3365=(
BOUNDED_SURFACE()
B_SPLINE_SURFACE(3,2,((#243136,#243137,#243138),(#243139,#243140,#243141),
(#243142,#243143,#243144),(#243145,#243146,#243147)),.UNSPECIFIED.,.F.,
 .F.,.F.)
B_SPLINE_SURFACE_WITH_KNOTS((4,4),(3,3),(-7.83336069620777E-18,0.000511815072430394),
(0.,1.00105598366044),.UNSPECIFIED.)
GEOMETRIC_REPRESENTATION_ITEM()
RATIONAL_B_SPLINE_SURFACE(((1.,0.706797490733229,1.00061923411797),(1.,
0.706182062146136,1.00062053388303),(1.,0.705584062768512,1.00062179683818),
(1.,0.705266224769987,1.00062246810164)))
REPRESENTATION_ITEM('')
SURFACE()
);
#3366=(
BOUNDED_SURFACE()
B_SPLINE_SURFACE(3,2,((#243153,#243154,#243155),(#243156,#243157,#243158),
(#243159,#243160,#243161),(#243162,#243163,#243164),(#243165,#243166,#243167),
(#243168,#243169,#243170)),.UNSPECIFIED.,.F.,.F.,.F.)
B_SPLINE_SURFACE_WITH_KNOTS((4,2,4),(3,3),(-5.42101086242752E-20,0.000257652232350883,
0.000515304464701767),(0.,1.),.UNSPECIFIED.)
GEOMETRIC_REPRESENTATION_ITEM()
RATIONAL_B_SPLINE_SURFACE(((1.,0.874619707139392,1.),(1.,0.874861180430363,
1.),(1.,0.855455725921355,1.),(1.,0.794699358954803,1.),(1.,0.753768977788994,
1.),(1.,0.708712527163659,1.)))
REPRESENTATION_ITEM('')
SURFACE()
);
#3367=(
BOUNDED_SURFACE()
B_SPLINE_SURFACE(3,2,((#243176,#243177,#243178),(#243179,#243180,#243181),
(#243182,#243183,#243184),(#243185,#243186,#243187)),.UNSPECIFIED.,.F.,
 .F.,.F.)
B_SPLINE_SURFACE_WITH_KNOTS((4,4),(3,3),(-5.42101086242752E-20,0.000397394373651941),
(0.,1.),.UNSPECIFIED.)
GEOMETRIC_REPRESENTATION_ITEM()
RATIONAL_B_SPLINE_SURFACE(((1.,0.707106781186548,1.),(1.,0.707752587915896,
1.),(1.,0.708377654540676,1.),(1.,0.708689770883328,1.)))
REPRESENTATION_ITEM('')
SURFACE()
);
#3368=(
BOUNDED_SURFACE()
B_SPLINE_SURFACE(3,2,((#243189,#243190,#243191),(#243192,#243193,#243194),
(#243195,#243196,#243197),(#243198,#243199,#243200)),.UNSPECIFIED.,.F.,
 .F.,.F.)
B_SPLINE_SURFACE_WITH_KNOTS((4,4),(3,3),(0.,0.000511815456479789),(0.,1.00105873159835),
 .UNSPECIFIED.)
GEOMETRIC_REPRESENTATION_ITEM()
RATIONAL_B_SPLINE_SURFACE(((1.,0.708394529056799,1.00061746385268),(1.,
0.708058564167347,1.00061817524597),(1.,0.707430835372527,1.00061950443859),
(1.,0.706796685880849,1.0006208472268)))
REPRESENTATION_ITEM('')
SURFACE()
);
#3369=(
BOUNDED_SURFACE()
B_SPLINE_SURFACE(3,2,((#243206,#243207,#243208),(#243209,#243210,#243211),
(#243212,#243213,#243214),(#243215,#243216,#243217)),.UNSPECIFIED.,.F.,
 .F.,.F.)
B_SPLINE_SURFACE_WITH_KNOTS((4,4),(3,3),(0.,0.000397394465448313),(0.,1.),
 .UNSPECIFIED.)
GEOMETRIC_REPRESENTATION_ITEM()
RATIONAL_B_SPLINE_SURFACE(((1.,0.705498956110762,1.),(1.,0.705821764811743,
1.),(1.,0.706461952521185,1.),(1.,0.707106781186556,1.)))
REPRESENTATION_ITEM('')
SURFACE()
);
#3370=(
BOUNDED_SURFACE()
B_SPLINE_SURFACE(3,2,((#243223,#243224,#243225),(#243226,#243227,#243228),
(#243229,#243230,#243231),(#243232,#243233,#243234)),.UNSPECIFIED.,.F.,
 .F.,.F.)
B_SPLINE_SURFACE_WITH_KNOTS((4,4),(3,3),(3.25260651745651E-18,0.000397394410828723),
(0.,1.),.UNSPECIFIED.)
GEOMETRIC_REPRESENTATION_ITEM()
RATIONAL_B_SPLINE_SURFACE(((1.,0.708689770883334,1.),(1.,0.708376440034478,
1.),(1.,0.707750498698416,1.),(1.,0.70710678118654,1.)))
REPRESENTATION_ITEM('')
SURFACE()
);
#3371=(
BOUNDED_SURFACE()
B_SPLINE_SURFACE(3,2,((#243240,#243241,#243242),(#243243,#243244,#243245),
(#243246,#243247,#243248),(#243249,#243250,#243251)),.UNSPECIFIED.,.F.,
 .F.,.F.)
B_SPLINE_SURFACE_WITH_KNOTS((4,4),(3,3),(-5.20417042793042E-18,0.00051181509012618),
(0.,1.00105592270183),.UNSPECIFIED.)
GEOMETRIC_REPRESENTATION_ITEM()
RATIONAL_B_SPLINE_SURFACE(((1.,0.705266242717577,1.00062243213062),(1.,
0.705584085909256,1.00062176089494),(1.,0.706182089450602,1.0006204980039),
(1.,0.706797508587584,1.00061919833383)))
REPRESENTATION_ITEM('')
SURFACE()
);
#3372=(
BOUNDED_SURFACE()
B_SPLINE_SURFACE(3,2,((#243253,#243254,#243255),(#243256,#243257,#243258),
(#243259,#243260,#243261),(#243262,#243263,#243264)),.UNSPECIFIED.,.F.,
 .F.,.F.)
B_SPLINE_SURFACE_WITH_KNOTS((4,4),(3,3),(0.,0.000397394428086615),(0.,1.),
 .UNSPECIFIED.)
GEOMETRIC_REPRESENTATION_ITEM()
RATIONAL_B_SPLINE_SURFACE(((1.,0.70710678118654,1.),(1.,0.706459846759078,
1.),(1.,0.705820510737278,1.),(1.,0.705498956110748,1.)))
REPRESENTATION_ITEM('')
SURFACE()
);
#3373=(
BOUNDED_SURFACE()
B_SPLINE_SURFACE(3,2,((#243270,#243271,#243272),(#243273,#243274,#243275),
(#243276,#243277,#243278),(#243279,#243280,#243281),(#243282,#243283,#243284),
(#243285,#243286,#243287)),.UNSPECIFIED.,.F.,.F.,.F.)
B_SPLINE_SURFACE_WITH_KNOTS((4,2,4),(3,3),(0.,0.000257953807872844,0.000515907615745689),
(0.,1.),.UNSPECIFIED.)
GEOMETRIC_REPRESENTATION_ITEM()
RATIONAL_B_SPLINE_SURFACE(((1.,0.874619707139402,1.),(1.,0.874834349679007,
1.),(1.,0.854686104157788,1.),(1.,0.792476597915144,1.),(1.,0.750887854595137,
1.),(1.,0.70558583803144,1.)))
REPRESENTATION_ITEM('')
SURFACE()
);
#3374=(
BOUNDED_SURFACE()
B_SPLINE_SURFACE(3,2,((#243293,#243294,#243295),(#243296,#243297,#243298),
(#243299,#243300,#243301),(#243302,#243303,#243304)),.UNSPECIFIED.,.F.,
 .F.,.F.)
B_SPLINE_SURFACE_WITH_KNOTS((4,4),(3,3),(-7.80625564189563E-18,0.000511815437699149),
(0.,1.00105881331508),.UNSPECIFIED.)
GEOMETRIC_REPRESENTATION_ITEM()
RATIONAL_B_SPLINE_SURFACE(((1.,0.706796661946571,1.00062089519671),(1.,
0.707430821225453,1.00061955228413),(1.,0.708058545830938,1.00061822299779),
(1.,0.708394505252939,1.00061751156117)))
REPRESENTATION_ITEM('')
SURFACE()
);
#3375=(
BOUNDED_SURFACE()
B_SPLINE_SURFACE(3,2,((#243306,#243307,#243308),(#243309,#243310,#243311),
(#243312,#243313,#243314),(#243315,#243316,#243317),(#243318,#243319,#243320),
(#243321,#243322,#243323)),.UNSPECIFIED.,.F.,.F.,.F.)
B_SPLINE_SURFACE_WITH_KNOTS((4,2,4),(3,3),(-2.87313575708659E-18,0.000256915317531263,
0.000513830635062528),(0.,1.),.UNSPECIFIED.)
GEOMETRIC_REPRESENTATION_ITEM()
RATIONAL_B_SPLINE_SURFACE(((1.,0.70558583803146,1.),(1.,0.750902433542788,
1.),(1.,0.792329530082522,1.),(1.,0.854288401594226,1.),(1.,0.874998031125156,
1.),(1.,0.874619707139415,1.)))
REPRESENTATION_ITEM('')
SURFACE()
);
#3376=(
BOUNDED_SURFACE()
B_SPLINE_SURFACE(3,2,((#243329,#243330,#243331),(#243332,#243333,#243334),
(#243335,#243336,#243337),(#243338,#243339,#243340),(#243341,#243342,#243343),
(#243344,#243345,#243346)),.UNSPECIFIED.,.F.,.F.,.F.)
B_SPLINE_SURFACE_WITH_KNOTS((4,2,4),(3,3),(-2.24971950790742E-18,0.000256592814262159,
0.00051318562852432),(0.,1.),.UNSPECIFIED.)
GEOMETRIC_REPRESENTATION_ITEM()
RATIONAL_B_SPLINE_SURFACE(((1.,0.708712527163664,1.),(1.,0.753780902613397,
1.),(1.,0.794538995769452,1.),(1.,0.85507077033087,1.),(1.,0.875018427445515,
1.),(1.,0.874619707139393,1.)))
REPRESENTATION_ITEM('')
SURFACE()
);
#3377=(
BOUNDED_SURFACE()
B_SPLINE_SURFACE(3,2,((#243348,#243349,#243350),(#243351,#243352,#243353),
(#243354,#243355,#243356),(#243357,#243358,#243359)),.UNSPECIFIED.,.F.,
 .F.,.F.)
B_SPLINE_SURFACE_WITH_KNOTS((4,4),(3,3),(-7.75204553327136E-18,0.000511815072430404),
(0.,1.00105598365717),.UNSPECIFIED.)
GEOMETRIC_REPRESENTATION_ITEM()
RATIONAL_B_SPLINE_SURFACE(((1.,0.70679749073418,1.00061923411605),(1.,0.706182062147123,
1.00062053388111),(1.,0.705584062769471,1.00062179683625),(1.,0.705266224770931,
1.00062246809971)))
REPRESENTATION_ITEM('')
SURFACE()
);
#3378=(
BOUNDED_SURFACE()
B_SPLINE_SURFACE(3,2,((#243365,#243366,#243367),(#243368,#243369,#243370),
(#243371,#243372,#243373),(#243374,#243375,#243376),(#243377,#243378,#243379),
(#243380,#243381,#243382)),.UNSPECIFIED.,.F.,.F.,.F.)
B_SPLINE_SURFACE_WITH_KNOTS((4,2,4),(3,3),(0.,0.000257652232350885,0.000515304464701769),
(0.,1.),.UNSPECIFIED.)
GEOMETRIC_REPRESENTATION_ITEM()
RATIONAL_B_SPLINE_SURFACE(((1.,0.874619707139384,1.),(1.,0.874861180430819,
1.),(1.,0.855455725920674,1.),(1.,0.794699358955418,1.),(1.,0.753768977788512,
1.),(1.,0.70871252716364,1.)))
REPRESENTATION_ITEM('')
SURFACE()
);
#3379=(
BOUNDED_SURFACE()
B_SPLINE_SURFACE(3,2,((#243388,#243389,#243390),(#243391,#243392,#243393),
(#243394,#243395,#243396),(#243397,#243398,#243399)),.UNSPECIFIED.,.F.,
 .F.,.F.)
B_SPLINE_SURFACE_WITH_KNOTS((4,4),(3,3),(-8.37546178245052E-18,0.000397394373651906),
(0.,1.),.UNSPECIFIED.)
GEOMETRIC_REPRESENTATION_ITEM()
RATIONAL_B_SPLINE_SURFACE(((1.,0.707106781186549,1.),(1.,0.707752587915899,
1.),(1.,0.708377654540661,1.),(1.,0.708689770883328,1.)))
REPRESENTATION_ITEM('')
SURFACE()
);
#3380=(
BOUNDED_SURFACE()
B_SPLINE_SURFACE(3,2,((#243401,#243402,#243403),(#243404,#243405,#243406),
(#243407,#243408,#243409),(#243410,#243411,#243412)),.UNSPECIFIED.,.F.,
 .F.,.F.)
B_SPLINE_SURFACE_WITH_KNOTS((4,4),(3,3),(0.,0.000511815456479786),(0.,1.00105873159754),
 .UNSPECIFIED.)
GEOMETRIC_REPRESENTATION_ITEM()
RATIONAL_B_SPLINE_SURFACE(((1.,0.708394529057023,1.00061746385221),(1.,
0.708058564167585,1.0006181752455),(1.,0.707430835372759,1.00061950443811),
(1.,0.706796685881085,1.00062084722632)))
REPRESENTATION_ITEM('')
SURFACE()
);
#3381=(
BOUNDED_SURFACE()
B_SPLINE_SURFACE(3,2,((#243418,#243419,#243420),(#243421,#243422,#243423),
(#243424,#243425,#243426),(#243427,#243428,#243429)),.UNSPECIFIED.,.F.,
 .F.,.F.)
B_SPLINE_SURFACE_WITH_KNOTS((4,4),(3,3),(-3.25260651745651E-18,0.000397394465448296),
(0.,1.),.UNSPECIFIED.)
GEOMETRIC_REPRESENTATION_ITEM()
RATIONAL_B_SPLINE_SURFACE(((1.,0.705498956110763,1.),(1.,0.705821764811817,
1.),(1.,0.70646195252111,1.),(1.,0.707106781186561,1.)))
REPRESENTATION_ITEM('')
SURFACE()
);
#3382=(
BOUNDED_SURFACE()
B_SPLINE_SURFACE(3,2,((#243435,#243436,#243437),(#243438,#243439,#243440),
(#243441,#243442,#243443),(#243444,#243445,#243446)),.UNSPECIFIED.,.F.,
 .F.,.F.)
B_SPLINE_SURFACE_WITH_KNOTS((4,4),(3,3),(0.,0.000397394410828747),(0.,1.),
 .UNSPECIFIED.)
GEOMETRIC_REPRESENTATION_ITEM()
RATIONAL_B_SPLINE_SURFACE(((1.,0.708689770883334,1.),(1.,0.708376440034482,
1.),(1.,0.707750498698421,1.),(1.,0.707106781186548,1.)))
REPRESENTATION_ITEM('')
SURFACE()
);
#3383=(
BOUNDED_SURFACE()
B_SPLINE_SURFACE(3,2,((#243452,#243453,#243454),(#243455,#243456,#243457),
(#243458,#243459,#243460),(#243461,#243462,#243463)),.UNSPECIFIED.,.F.,
 .F.,.F.)
B_SPLINE_SURFACE_WITH_KNOTS((4,4),(3,3),(0.,0.000511815090126157),(0.,1.00105592270313),
 .UNSPECIFIED.)
GEOMETRIC_REPRESENTATION_ITEM()
RATIONAL_B_SPLINE_SURFACE(((1.,0.705266242717223,1.00062243213138),(1.,
0.705584085908876,1.0006217608957),(1.,0.706182089450213,1.00062049800467),
(1.,0.706797508587211,1.00061919833459)))
REPRESENTATION_ITEM('')
SURFACE()
);
#3384=(
BOUNDED_SURFACE()
B_SPLINE_SURFACE(3,2,((#243465,#243466,#243467),(#243468,#243469,#243470),
(#243471,#243472,#243473),(#243474,#243475,#243476)),.UNSPECIFIED.,.F.,
 .F.,.F.)
B_SPLINE_SURFACE_WITH_KNOTS((4,4),(3,3),(0.,0.000397394428086609),(0.,1.),
 .UNSPECIFIED.)
GEOMETRIC_REPRESENTATION_ITEM()
RATIONAL_B_SPLINE_SURFACE(((1.,0.707106781186544,1.),(1.,0.706459846759089,
1.),(1.,0.705820510737274,1.),(1.,0.705498956110742,1.)))
REPRESENTATION_ITEM('')
SURFACE()
);
#3385=(
BOUNDED_SURFACE()
B_SPLINE_SURFACE(3,2,((#243482,#243483,#243484),(#243485,#243486,#243487),
(#243488,#243489,#243490),(#243491,#243492,#243493),(#243494,#243495,#243496),
(#243497,#243498,#243499)),.UNSPECIFIED.,.F.,.F.,.F.)
B_SPLINE_SURFACE_WITH_KNOTS((4,2,4),(3,3),(0.,0.000257953807872844,0.000515907615745688),
(0.,1.),.UNSPECIFIED.)
GEOMETRIC_REPRESENTATION_ITEM()
RATIONAL_B_SPLINE_SURFACE(((1.,0.874619707139395,1.),(1.,0.874834349678822,
1.),(1.,0.854686104158037,1.),(1.,0.792476597914894,1.),(1.,0.750887854595317,
1.),(1.,0.705585838031437,1.)))
REPRESENTATION_ITEM('')
SURFACE()
);
#3386=(
BOUNDED_SURFACE()
B_SPLINE_SURFACE(3,2,((#243505,#243506,#243507),(#243508,#243509,#243510),
(#243511,#243512,#243513),(#243514,#243515,#243516)),.UNSPECIFIED.,.F.,
 .F.,.F.)
B_SPLINE_SURFACE_WITH_KNOTS((4,4),(3,3),(-6.7762635780344E-19,0.000511815437699156),
(0.,1.00105881331755),.UNSPECIFIED.)
GEOMETRIC_REPRESENTATION_ITEM()
RATIONAL_B_SPLINE_SURFACE(((1.,0.706796661945847,1.00062089519816),(1.,
0.707430821224722,1.00061955228558),(1.,0.708058545830208,1.00061822299924),
(1.,0.708394505252233,1.00061751156262)))
REPRESENTATION_ITEM('')
SURFACE()
);
#3387=(
BOUNDED_SURFACE()
B_SPLINE_SURFACE(3,2,((#243518,#243519,#243520),(#243521,#243522,#243523),
(#243524,#243525,#243526),(#243527,#243528,#243529),(#243530,#243531,#243532),
(#243533,#243534,#243535)),.UNSPECIFIED.,.F.,.F.,.F.)
B_SPLINE_SURFACE_WITH_KNOTS((4,2,4),(3,3),(-2.71050543121376E-20,0.000256915317531267,
0.000513830635062534),(0.,1.),.UNSPECIFIED.)
GEOMETRIC_REPRESENTATION_ITEM()
RATIONAL_B_SPLINE_SURFACE(((1.,0.705585838031452,1.),(1.,0.750902433542858,
1.),(1.,0.792329530082393,1.),(1.,0.854288401594359,1.),(1.,0.874998031125022,
1.),(1.,0.874619707139412,1.)))
REPRESENTATION_ITEM('')
SURFACE()
);
#3388=(
BOUNDED_SURFACE()
B_SPLINE_SURFACE(3,2,((#243541,#243542,#243543),(#243544,#243545,#243546),
(#243547,#243548,#243549),(#243550,#243551,#243552),(#243553,#243554,#243555),
(#243556,#243557,#243558)),.UNSPECIFIED.,.F.,.F.,.F.)
B_SPLINE_SURFACE_WITH_KNOTS((4,2,4),(3,3),(0.,0.00025659281426216,0.00051318562852432),
(0.,1.),.UNSPECIFIED.)
GEOMETRIC_REPRESENTATION_ITEM()
RATIONAL_B_SPLINE_SURFACE(((1.,0.708712527163661,1.),(1.,0.753780902613585,
1.),(1.,0.794538995769198,1.),(1.,0.855070770331121,1.),(1.,0.875018427445309,
1.),(1.,0.874619707139393,1.)))
REPRESENTATION_ITEM('')
SURFACE()
);
#3389=(
BOUNDED_SURFACE()
B_SPLINE_SURFACE(3,2,((#243560,#243561,#243562),(#243563,#243564,#243565),
(#243566,#243567,#243568),(#243569,#243570,#243571)),.UNSPECIFIED.,.F.,
 .F.,.F.)
B_SPLINE_SURFACE_WITH_KNOTS((4,4),(3,3),(5.96311194867027E-19,0.000511815072430393),
(0.,1.00105598365635),.UNSPECIFIED.)
GEOMETRIC_REPRESENTATION_ITEM()
RATIONAL_B_SPLINE_SURFACE(((1.,0.706797490734424,1.00061923411557),(1.,
0.706182062147336,1.00062053388063),(1.,0.705584062769713,1.00062179683577),
(1.,0.705266224771183,1.00062246809923)))
REPRESENTATION_ITEM('')
SURFACE()
);
#3390=(
BOUNDED_SURFACE()
B_SPLINE_SURFACE(3,2,((#243577,#243578,#243579),(#243580,#243581,#243582),
(#243583,#243584,#243585),(#243586,#243587,#243588),(#243589,#243590,#243591),
(#243592,#243593,#243594)),.UNSPECIFIED.,.F.,.F.,.F.)
B_SPLINE_SURFACE_WITH_KNOTS((4,2,4),(3,3),(0.,0.000257652232350886,0.000515304464701771),
(0.,1.),.UNSPECIFIED.)
GEOMETRIC_REPRESENTATION_ITEM()
RATIONAL_B_SPLINE_SURFACE(((1.,0.874619707139397,1.),(1.,0.874861180431091,
1.),(1.,0.85545572592034,1.),(1.,0.794699358955775,1.),(1.,0.75376897778827,
1.),(1.,0.708712527163653,1.)))
REPRESENTATION_ITEM('')
SURFACE()
);
#3391=(
BOUNDED_SURFACE()
B_SPLINE_SURFACE(3,2,((#243600,#243601,#243602),(#243603,#243604,#243605),
(#243606,#243607,#243608),(#243609,#243610,#243611)),.UNSPECIFIED.,.F.,
 .F.,.F.)
B_SPLINE_SURFACE_WITH_KNOTS((4,4),(3,3),(0.,0.000397394373651917),(0.,1.),
 .UNSPECIFIED.)
GEOMETRIC_REPRESENTATION_ITEM()
RATIONAL_B_SPLINE_SURFACE(((1.,0.707106781186548,1.),(1.,0.707752587915883,
1.),(1.,0.708377654540707,1.),(1.,0.70868977088332,1.)))
REPRESENTATION_ITEM('')
SURFACE()
);
#3392=(
BOUNDED_SURFACE()
B_SPLINE_SURFACE(3,2,((#243613,#243614,#243615),(#243616,#243617,#243618),
(#243619,#243620,#243621),(#243622,#243623,#243624)),.UNSPECIFIED.,.F.,
 .F.,.F.)
B_SPLINE_SURFACE_WITH_KNOTS((4,4),(3,3),(-8.02309607639273E-18,0.000511815456479797),
(0.,1.0010587315978),.UNSPECIFIED.)
GEOMETRIC_REPRESENTATION_ITEM()
RATIONAL_B_SPLINE_SURFACE(((1.,0.708394529056956,1.00061746385236),(1.,
0.708058564167499,1.00061817524565),(1.,0.707430835372702,1.00061950443827),
(1.,0.706796685881003,1.00062084722648)))
REPRESENTATION_ITEM('')
SURFACE()
);
#3393=(
BOUNDED_SURFACE()
B_SPLINE_SURFACE(3,2,((#243630,#243631,#243632),(#243633,#243634,#243635),
(#243636,#243637,#243638),(#243639,#243640,#243641)),.UNSPECIFIED.,.F.,
 .F.,.F.)
B_SPLINE_SURFACE_WITH_KNOTS((4,4),(3,3),(0.,0.000397394465448314),(0.,1.),
 .UNSPECIFIED.)
GEOMETRIC_REPRESENTATION_ITEM()
RATIONAL_B_SPLINE_SURFACE(((1.,0.705498956110746,1.),(1.,0.705821764811783,
1.),(1.,0.706461952521148,1.),(1.,0.707106781186544,1.)))
REPRESENTATION_ITEM('')
SURFACE()
);
#3394=(
BOUNDED_SURFACE()
B_SPLINE_SURFACE(3,2,((#243647,#243648,#243649),(#243650,#243651,#243652),
(#243653,#243654,#243655),(#243656,#243657,#243658)),.UNSPECIFIED.,.F.,
 .F.,.F.)
B_SPLINE_SURFACE_WITH_KNOTS((4,4),(3,3),(0.,0.000397394410828735),(0.,1.),
 .UNSPECIFIED.)
GEOMETRIC_REPRESENTATION_ITEM()
RATIONAL_B_SPLINE_SURFACE(((1.,0.708689770883323,1.),(1.,0.708376440034487,
1.),(1.,0.707750498698403,1.),(1.,0.707106781186548,1.)))
REPRESENTATION_ITEM('')
SURFACE()
);
#3395=(
BOUNDED_SURFACE()
B_SPLINE_SURFACE(3,2,((#243664,#243665,#243666),(#243667,#243668,#243669),
(#243670,#243671,#243672),(#243673,#243674,#243675)),.UNSPECIFIED.,.F.,
 .F.,.F.)
B_SPLINE_SURFACE_WITH_KNOTS((4,4),(3,3),(0.,0.000511815090126168),(0.,1.00105592270543),
 .UNSPECIFIED.)
GEOMETRIC_REPRESENTATION_ITEM()
RATIONAL_B_SPLINE_SURFACE(((1.,0.70526624271654,1.00062243213275),(1.,0.705584085908197,
1.00062176089706),(1.,0.706182089449555,1.00062049800603),(1.,0.706797508586535,
1.00061919833595)))
REPRESENTATION_ITEM('')
SURFACE()
);
#3396=(
BOUNDED_SURFACE()
B_SPLINE_SURFACE(3,2,((#243677,#243678,#243679),(#243680,#243681,#243682),
(#243683,#243684,#243685),(#243686,#243687,#243688)),.UNSPECIFIED.,.F.,
 .F.,.F.)
B_SPLINE_SURFACE_WITH_KNOTS((4,4),(3,3),(0.,0.000397394428086615),(0.,1.),
 .UNSPECIFIED.)
GEOMETRIC_REPRESENTATION_ITEM()
RATIONAL_B_SPLINE_SURFACE(((1.,0.707106781186548,1.),(1.,0.706459846759084,
1.),(1.,0.705820510737294,1.),(1.,0.705498956110758,1.)))
REPRESENTATION_ITEM('')
SURFACE()
);
#3397=(
BOUNDED_SURFACE()
B_SPLINE_SURFACE(3,2,((#243694,#243695,#243696),(#243697,#243698,#243699),
(#243700,#243701,#243702),(#243703,#243704,#243705),(#243706,#243707,#243708),
(#243709,#243710,#243711)),.UNSPECIFIED.,.F.,.F.,.F.)
B_SPLINE_SURFACE_WITH_KNOTS((4,2,4),(3,3),(-3.93023287525995E-19,0.000257953807872852,
0.000515907615745705),(0.,1.),.UNSPECIFIED.)
GEOMETRIC_REPRESENTATION_ITEM()
RATIONAL_B_SPLINE_SURFACE(((1.,0.874619707139391,1.),(1.,0.874834349678696,
1.),(1.,0.854686104158193,1.),(1.,0.792476597914731,1.),(1.,0.750887854595441,
1.),(1.,0.705585838031444,1.)))
REPRESENTATION_ITEM('')
SURFACE()
);
#3398=(
BOUNDED_SURFACE()
B_SPLINE_SURFACE(3,2,((#243717,#243718,#243719),(#243720,#243721,#243722),
(#243723,#243724,#243725),(#243726,#243727,#243728)),.UNSPECIFIED.,.F.,
 .F.,.F.)
B_SPLINE_SURFACE_WITH_KNOTS((4,4),(3,3),(-5.6920614055489E-19,0.000511815437699152),
(0.,1.00105881331654),.UNSPECIFIED.)
GEOMETRIC_REPRESENTATION_ITEM()
RATIONAL_B_SPLINE_SURFACE(((1.,0.706796661946145,1.00062089519757),(1.,
0.707430821225015,1.00061955228499),(1.,0.708058545830515,1.00061822299865),
(1.,0.70839450525252,1.00061751156203)))
REPRESENTATION_ITEM('')
SURFACE()
);
#3399=(
BOUNDED_SURFACE()
B_SPLINE_SURFACE(3,2,((#243730,#243731,#243732),(#243733,#243734,#243735),
(#243736,#243737,#243738),(#243739,#243740,#243741),(#243742,#243743,#243744),
(#243745,#243746,#243747)),.UNSPECIFIED.,.F.,.F.,.F.)
B_SPLINE_SURFACE_WITH_KNOTS((4,2,4),(3,3),(-2.7376104855259E-18,0.000256915317531256,
0.000513830635062514),(0.,1.),.UNSPECIFIED.)
GEOMETRIC_REPRESENTATION_ITEM()
RATIONAL_B_SPLINE_SURFACE(((1.,0.705585838031416,1.),(1.,0.750902433542311,
1.),(1.,0.792329530083129,1.),(1.,0.854288401593573,1.),(1.,0.874998031125583,
1.),(1.,0.874619707139392,1.)))
REPRESENTATION_ITEM('')
SURFACE()
);
#3400=(
BOUNDED_SURFACE()
B_SPLINE_SURFACE(3,2,((#243753,#243754,#243755),(#243756,#243757,#243758),
(#243759,#243760,#243761),(#243762,#243763,#243764),(#243765,#243766,#243767),
(#243768,#243769,#243770)),.UNSPECIFIED.,.F.,.F.,.F.)
B_SPLINE_SURFACE_WITH_KNOTS((4,2,4),(3,3),(0.,0.000256592814262159,0.000513185628524319),
(0.,1.),.UNSPECIFIED.)
GEOMETRIC_REPRESENTATION_ITEM()
RATIONAL_B_SPLINE_SURFACE(((1.,0.708712527163655,1.),(1.,0.753780902613272,
1.),(1.,0.794538995769632,1.),(1.,0.855070770330658,1.),(1.,0.875018427445671,
1.),(1.,0.874619707139395,1.)))
REPRESENTATION_ITEM('')
SURFACE()
);
#3401=(
BOUNDED_SURFACE()
B_SPLINE_SURFACE(3,2,((#243772,#243773,#243774),(#243775,#243776,#243777),
(#243778,#243779,#243780),(#243781,#243782,#243783)),.UNSPECIFIED.,.F.,
 .F.,.F.)
B_SPLINE_SURFACE_WITH_KNOTS((4,4),(3,3),(5.6920614055489E-19,0.000511815072430395),
(0.,1.00105598365956),.UNSPECIFIED.)
GEOMETRIC_REPRESENTATION_ITEM()
RATIONAL_B_SPLINE_SURFACE(((1.,0.706797490733483,1.00061923411746),(1.,
0.706182062146394,1.00062053388252),(1.,0.705584062768761,1.00062179683766),
(1.,0.705266224770235,1.00062246810113)))
REPRESENTATION_ITEM('')
SURFACE()
);
#3402=(
BOUNDED_SURFACE()
B_SPLINE_SURFACE(3,2,((#243789,#243790,#243791),(#243792,#243793,#243794),
(#243795,#243796,#243797),(#243798,#243799,#243800),(#243801,#243802,#243803),
(#243804,#243805,#243806)),.UNSPECIFIED.,.F.,.F.,.F.)
B_SPLINE_SURFACE_WITH_KNOTS((4,2,4),(3,3),(0.,0.000257652232350885,0.00051530446470177),
(0.,1.),.UNSPECIFIED.)
GEOMETRIC_REPRESENTATION_ITEM()
RATIONAL_B_SPLINE_SURFACE(((1.,0.8746197071394,1.),(1.,0.874861180430967,
1.),(1.,0.85545572592054,1.),(1.,0.794699358955578,1.),(1.,0.753768977788408,
1.),(1.,0.708712527163672,1.)))
REPRESENTATION_ITEM('')
SURFACE()
);
#3403=(
BOUNDED_SURFACE()
B_SPLINE_SURFACE(3,2,((#243812,#243813,#243814),(#243815,#243816,#243817),
(#243818,#243819,#243820),(#243821,#243822,#243823)),.UNSPECIFIED.,.F.,
 .F.,.F.)
B_SPLINE_SURFACE_WITH_KNOTS((4,4),(3,3),(-7.10152422978005E-18,0.00039739437365192),
(0.,1.),.UNSPECIFIED.)
GEOMETRIC_REPRESENTATION_ITEM()
RATIONAL_B_SPLINE_SURFACE(((1.,0.707106781186545,1.),(1.,0.707752587915908,
1.),(1.,0.708377654540671,1.),(1.,0.708689770883337,1.)))
REPRESENTATION_ITEM('')
SURFACE()
);
#3404=(
BOUNDED_SURFACE()
B_SPLINE_SURFACE(3,2,((#243825,#243826,#243827),(#243828,#243829,#243830),
(#243831,#243832,#243833),(#243834,#243835,#243836)),.UNSPECIFIED.,.F.,
 .F.,.F.)
B_SPLINE_SURFACE_WITH_KNOTS((4,4),(3,3),(0.,0.000511815456479799),(0.,1.00105873159959),
 .UNSPECIFIED.)
GEOMETRIC_REPRESENTATION_ITEM()
RATIONAL_B_SPLINE_SURFACE(((1.,0.70839452905644,1.0006174638534),(1.,0.708058564166983,
1.00061817524669),(1.,0.707430835372161,1.00061950443932),(1.,0.706796685880483,
1.00062084722753)))
REPRESENTATION_ITEM('')
SURFACE()
);
#3405=(
BOUNDED_SURFACE()
B_SPLINE_SURFACE(3,2,((#243842,#243843,#243844),(#243845,#243846,#243847),
(#243848,#243849,#243850),(#243851,#243852,#243853)),.UNSPECIFIED.,.F.,
 .F.,.F.)
B_SPLINE_SURFACE_WITH_KNOTS((4,4),(3,3),(-5.6920614055489E-18,0.000397394465448304),
(0.,1.),.UNSPECIFIED.)
GEOMETRIC_REPRESENTATION_ITEM()
RATIONAL_B_SPLINE_SURFACE(((1.,0.705498956110744,1.),(1.,0.705821764811792,
1.),(1.,0.706461952521134,1.),(1.,0.707106781186545,1.)))
REPRESENTATION_ITEM('')
SURFACE()
);
#3406=(
BOUNDED_SURFACE()
B_SPLINE_SURFACE(3,2,((#243859,#243860,#243861),(#243862,#243863,#243864),
(#243865,#243866,#243867),(#243868,#243869,#243870)),.UNSPECIFIED.,.F.,
 .F.,.F.)
B_SPLINE_SURFACE_WITH_KNOTS((4,4),(3,3),(0.,0.00039739441082873),(0.,1.),
 .UNSPECIFIED.)
GEOMETRIC_REPRESENTATION_ITEM()
RATIONAL_B_SPLINE_SURFACE(((1.,0.708689770883332,1.),(1.,0.70837644003449,
1.),(1.,0.707750498698411,1.),(1.,0.707106781186548,1.)))
REPRESENTATION_ITEM('')
SURFACE()
);
#3407=(
BOUNDED_SURFACE()
B_SPLINE_SURFACE(3,2,((#243876,#243877,#243878),(#243879,#243880,#243881),
(#243882,#243883,#243884),(#243885,#243886,#243887)),.UNSPECIFIED.,.F.,
 .F.,.F.)
B_SPLINE_SURFACE_WITH_KNOTS((4,4),(3,3),(0.,0.000511815090126174),(0.,1.00105592270389),
 .UNSPECIFIED.)
GEOMETRIC_REPRESENTATION_ITEM()
RATIONAL_B_SPLINE_SURFACE(((1.,0.70526624271697,1.00062243213183),(1.,0.705584085908647,
1.00062176089615),(1.,0.706182089450001,1.00062049800512),(1.,0.706797508586988,
1.00061919833504)))
REPRESENTATION_ITEM('')
SURFACE()
);
#3408=(
BOUNDED_SURFACE()
B_SPLINE_SURFACE(3,2,((#243889,#243890,#243891),(#243892,#243893,#243894),
(#243895,#243896,#243897),(#243898,#243899,#243900)),.UNSPECIFIED.,.F.,
 .F.,.F.)
B_SPLINE_SURFACE_WITH_KNOTS((4,4),(3,3),(-7.07441917546792E-18,0.00039739442808661),
(0.,1.),.UNSPECIFIED.)
GEOMETRIC_REPRESENTATION_ITEM()
RATIONAL_B_SPLINE_SURFACE(((1.,0.707106781186547,1.),(1.,0.706459846759101,
1.),(1.,0.705820510737253,1.),(1.,0.705498956110768,1.)))
REPRESENTATION_ITEM('')
SURFACE()
);
#3409=(
BOUNDED_SURFACE()
B_SPLINE_SURFACE(3,2,((#243906,#243907,#243908),(#243909,#243910,#243911),
(#243912,#243913,#243914),(#243915,#243916,#243917),(#243918,#243919,#243920),
(#243921,#243922,#243923)),.UNSPECIFIED.,.F.,.F.,.F.)
B_SPLINE_SURFACE_WITH_KNOTS((4,2,4),(3,3),(0.,0.000257953807872856,0.000515907615745713),
(0.,1.),.UNSPECIFIED.)
GEOMETRIC_REPRESENTATION_ITEM()
RATIONAL_B_SPLINE_SURFACE(((1.,0.874619707139396,1.),(1.,0.874834349678934,
1.),(1.,0.85468610415787,1.),(1.,0.79247659791506,1.),(1.,0.750887854595183,
1.),(1.,0.70558583803143,1.)))
REPRESENTATION_ITEM('')
SURFACE()
);
#3410=(
BOUNDED_SURFACE()
B_SPLINE_SURFACE(3,2,((#243929,#243930,#243931),(#243932,#243933,#243934),
(#243935,#243936,#243937),(#243938,#243939,#243940)),.UNSPECIFIED.,.F.,
 .F.,.F.)
B_SPLINE_SURFACE_WITH_KNOTS((4,4),(3,3),(0.,0.00051181543769915),(0.,1.00105881331475),
 .UNSPECIFIED.)
GEOMETRIC_REPRESENTATION_ITEM()
RATIONAL_B_SPLINE_SURFACE(((1.,0.706796661946667,1.00062089519652),(1.,
0.70743082122554,1.00061955228395),(1.,0.708058545831051,1.0006182229976),
(1.,0.708394505253048,1.00061751156099)))
REPRESENTATION_ITEM('')
SURFACE()
);
#3411=(
BOUNDED_SURFACE()
B_SPLINE_SURFACE(3,2,((#243942,#243943,#243944),(#243945,#243946,#243947),
(#243948,#243949,#243950),(#243951,#243952,#243953),(#243954,#243955,#243956),
(#243957,#243958,#243959)),.UNSPECIFIED.,.F.,.F.,.F.)
B_SPLINE_SURFACE_WITH_KNOTS((4,2,4),(3,3),(-2.71050543121376E-20,0.000256915317531261,
0.000513830635062521),(0.,1.),.UNSPECIFIED.)
GEOMETRIC_REPRESENTATION_ITEM()
RATIONAL_B_SPLINE_SURFACE(((1.,0.705585838031441,1.),(1.,0.750902433542888,
1.),(1.,0.792329530082332,1.),(1.,0.854288401594382,1.),(1.,0.874998031124998,
1.),(1.,0.874619707139396,1.)))
REPRESENTATION_ITEM('')
SURFACE()
);
#3412=(
BOUNDED_SURFACE()
B_SPLINE_SURFACE(3,2,((#243965,#243966,#243967),(#243968,#243969,#243970),
(#243971,#243972,#243973),(#243974,#243975,#243976),(#243977,#243978,#243979),
(#243980,#243981,#243982)),.UNSPECIFIED.,.F.,.F.,.F.)
B_SPLINE_SURFACE_WITH_KNOTS((4,2,4),(3,3),(-1.0435445910173E-17,0.000256592814262151,
0.000513185628524313),(0.,1.),.UNSPECIFIED.)
GEOMETRIC_REPRESENTATION_ITEM()
RATIONAL_B_SPLINE_SURFACE(((1.,0.70871252716368,1.),(1.,0.753780902613545,
1.),(1.,0.794538995769243,1.),(1.,0.855070770331071,1.),(1.,0.875018427445353,
1.),(1.,0.874619707139393,1.)))
REPRESENTATION_ITEM('')
SURFACE()
);
#3413=(
BOUNDED_SURFACE()
B_SPLINE_SURFACE(3,2,((#243984,#243985,#243986),(#243987,#243988,#243989),
(#243990,#243991,#243992),(#243993,#243994,#243995)),.UNSPECIFIED.,.F.,
 .F.,.F.)
B_SPLINE_SURFACE_WITH_KNOTS((4,4),(3,3),(5.6920614055489E-19,0.000511815072430399),
(0.,1.00105598365992),.UNSPECIFIED.)
GEOMETRIC_REPRESENTATION_ITEM()
RATIONAL_B_SPLINE_SURFACE(((1.,0.70679749073338,1.00061923411767),(1.,0.706182062146294,
1.00062053388273),(1.,0.70558406276866,1.00062179683787),(1.,0.705266224770139,
1.00062246810134)))
REPRESENTATION_ITEM('')
SURFACE()
);
#3414=(
BOUNDED_SURFACE()
B_SPLINE_SURFACE(3,2,((#244001,#244002,#244003),(#244004,#244005,#244006),
(#244007,#244008,#244009),(#244010,#244011,#244012),(#244013,#244014,#244015),
(#244016,#244017,#244018)),.UNSPECIFIED.,.F.,.F.,.F.)
B_SPLINE_SURFACE_WITH_KNOTS((4,2,4),(3,3),(-6.36968776335234E-19,0.000257652232350878,
0.000515304464701757),(0.,1.),.UNSPECIFIED.)
GEOMETRIC_REPRESENTATION_ITEM()
RATIONAL_B_SPLINE_SURFACE(((1.,0.874619707139393,1.),(1.,0.874861180431038,
1.),(1.,0.855455725920423,1.),(1.,0.794699358955735,1.),(1.,0.753768977788282,
1.),(1.,0.708712527163677,1.)))
REPRESENTATION_ITEM('')
SURFACE()
);
#3415=(
BOUNDED_SURFACE()
B_SPLINE_SURFACE(3,2,((#244024,#244025,#244026),(#244027,#244028,#244029),
(#244030,#244031,#244032),(#244033,#244034,#244035)),.UNSPECIFIED.,.F.,
 .F.,.F.)
B_SPLINE_SURFACE_WITH_KNOTS((4,4),(3,3),(0.,0.000397394373651921),(0.,1.),
 .UNSPECIFIED.)
GEOMETRIC_REPRESENTATION_ITEM()
RATIONAL_B_SPLINE_SURFACE(((1.,0.707106781186548,1.),(1.,0.707752587915887,
1.),(1.,0.708377654540684,1.),(1.,0.70868977088333,1.)))
REPRESENTATION_ITEM('')
SURFACE()
);
#3416=(
BOUNDED_SURFACE()
B_SPLINE_SURFACE(3,2,((#244037,#244038,#244039),(#244040,#244041,#244042),
(#244043,#244044,#244045),(#244046,#244047,#244048)),.UNSPECIFIED.,.F.,
 .F.,.F.)
B_SPLINE_SURFACE_WITH_KNOTS((4,4),(3,3),(0.,0.0005118154564798),(0.,1.0010587315969),
 .UNSPECIFIED.)
GEOMETRIC_REPRESENTATION_ITEM()
RATIONAL_B_SPLINE_SURFACE(((1.,0.708394529057217,1.00061746385183),(1.,
0.70805856416776,1.00061817524512),(1.,0.707430835372961,1.00061950443774),
(1.,0.706796685881273,1.00062084722595)))
REPRESENTATION_ITEM('')
SURFACE()
);
#3417=(
BOUNDED_SURFACE()
B_SPLINE_SURFACE(3,2,((#244054,#244055,#244056),(#244057,#244058,#244059),
(#244060,#244061,#244062),(#244063,#244064,#244065)),.UNSPECIFIED.,.F.,
 .F.,.F.)
B_SPLINE_SURFACE_WITH_KNOTS((4,4),(3,3),(-2.03287907341032E-18,0.000397394465448303),
(0.,1.),.UNSPECIFIED.)
GEOMETRIC_REPRESENTATION_ITEM()
RATIONAL_B_SPLINE_SURFACE(((1.,0.705498956110753,1.),(1.,0.705821764811784,
1.),(1.,0.706461952521139,1.),(1.,0.707106781186548,1.)))
REPRESENTATION_ITEM('')
SURFACE()
);
#3418=(
BOUNDED_SURFACE()
B_SPLINE_SURFACE(3,2,((#244071,#244072,#244073),(#244074,#244075,#244076),
(#244077,#244078,#244079),(#244080,#244081,#244082)),.UNSPECIFIED.,.F.,
 .F.,.F.)
B_SPLINE_SURFACE_WITH_KNOTS((4,4),(3,3),(0.,0.000397394410828748),(0.,1.),
 .UNSPECIFIED.)
GEOMETRIC_REPRESENTATION_ITEM()
RATIONAL_B_SPLINE_SURFACE(((1.,0.708689770883308,1.),(1.,0.708376440034495,
1.),(1.,0.707750498698405,1.),(1.,0.707106781186549,1.)))
REPRESENTATION_ITEM('')
SURFACE()
);
#3419=(
BOUNDED_SURFACE()
B_SPLINE_SURFACE(3,2,((#244088,#244089,#244090),(#244091,#244092,#244093),
(#244094,#244095,#244096),(#244097,#244098,#244099)),.UNSPECIFIED.,.F.,
 .F.,.F.)
B_SPLINE_SURFACE_WITH_KNOTS((4,4),(3,3),(0.,0.000511815090126176),(0.,1.00105592270268),
 .UNSPECIFIED.)
GEOMETRIC_REPRESENTATION_ITEM()
RATIONAL_B_SPLINE_SURFACE(((1.,0.705266242717368,1.00062243213112),(1.,
0.705584085908997,1.00062176089544),(1.,0.706182089450358,1.00062049800441),
(1.,0.706797508587342,1.00061919833433)))
REPRESENTATION_ITEM('')
SURFACE()
);
#3420=(
BOUNDED_SURFACE()
B_SPLINE_SURFACE(3,2,((#244101,#244102,#244103),(#244104,#244105,#244106),
(#244107,#244108,#244109),(#244110,#244111,#244112)),.UNSPECIFIED.,.F.,
 .F.,.F.)
B_SPLINE_SURFACE_WITH_KNOTS((4,4),(3,3),(0.,0.000397394428086627),(0.,1.),
 .UNSPECIFIED.)
GEOMETRIC_REPRESENTATION_ITEM()
RATIONAL_B_SPLINE_SURFACE(((1.,0.70710678118655,1.),(1.,0.706459846759099,
1.),(1.,0.705820510737279,1.),(1.,0.70549895611076,1.)))
REPRESENTATION_ITEM('')
SURFACE()
);
#3421=(
BOUNDED_SURFACE()
B_SPLINE_SURFACE(3,2,((#244118,#244119,#244120),(#244121,#244122,#244123),
(#244124,#244125,#244126),(#244127,#244128,#244129),(#244130,#244131,#244132),
(#244133,#244134,#244135)),.UNSPECIFIED.,.F.,.F.,.F.)
B_SPLINE_SURFACE_WITH_KNOTS((4,2,4),(3,3),(0.,0.000257953807872846,0.000515907615745692),
(0.,1.),.UNSPECIFIED.)
GEOMETRIC_REPRESENTATION_ITEM()
RATIONAL_B_SPLINE_SURFACE(((1.,0.874619707139392,1.),(1.,0.874834349678668,
1.),(1.,0.854686104158253,1.),(1.,0.792476597914677,1.),(1.,0.750887854595503,
1.),(1.,0.705585838031432,1.)))
REPRESENTATION_ITEM('')
SURFACE()
);
#3422=(
BOUNDED_SURFACE()
B_SPLINE_SURFACE(3,2,((#244141,#244142,#244143),(#244144,#244145,#244146),
(#244147,#244148,#244149),(#244150,#244151,#244152)),.UNSPECIFIED.,.F.,
 .F.,.F.)
B_SPLINE_SURFACE_WITH_KNOTS((4,4),(3,3),(-5.6920614055489E-19,0.00051181543769915),
(0.,1.0010588133166),.UNSPECIFIED.)
GEOMETRIC_REPRESENTATION_ITEM()
RATIONAL_B_SPLINE_SURFACE(((1.,0.706796661946126,1.00062089519761),(1.,
0.707430821224993,1.00061955228503),(1.,0.708058545830525,1.00061822299868),
(1.,0.708394505252487,1.00061751156206)))
REPRESENTATION_ITEM('')
SURFACE()
);
#3423=(
BOUNDED_SURFACE()
B_SPLINE_SURFACE(3,2,((#244154,#244155,#244156),(#244157,#244158,#244159),
(#244160,#244161,#244162),(#244163,#244164,#244165),(#244166,#244167,#244168),
(#244169,#244170,#244171)),.UNSPECIFIED.,.F.,.F.,.F.)
B_SPLINE_SURFACE_WITH_KNOTS((4,2,4),(3,3),(0.,0.000256915317531263,0.000513830635062526),
(0.,1.),.UNSPECIFIED.)
GEOMETRIC_REPRESENTATION_ITEM()
RATIONAL_B_SPLINE_SURFACE(((1.,0.705585838031459,1.),(1.,0.750902433542461,
1.),(1.,0.79232953008286,1.),(1.,0.854288401593831,1.),(1.,0.874998031125431,
1.),(1.,0.87461970713939,1.)))
REPRESENTATION_ITEM('')
SURFACE()
);
#3424=(
BOUNDED_SURFACE()
B_SPLINE_SURFACE(3,2,((#244177,#244178,#244179),(#244180,#244181,#244182),
(#244183,#244184,#244185),(#244186,#244187,#244188),(#244189,#244190,#244191),
(#244192,#244193,#244194)),.UNSPECIFIED.,.F.,.F.,.F.)
B_SPLINE_SURFACE_WITH_KNOTS((4,2,4),(3,3),(0.,0.000256592814262157,0.000513185628524313),
(0.,1.),.UNSPECIFIED.)
GEOMETRIC_REPRESENTATION_ITEM()
RATIONAL_B_SPLINE_SURFACE(((1.,0.708712527163657,1.),(1.,0.753780902614056,
1.),(1.,0.794538995768585,1.),(1.,0.855070770331729,1.),(1.,0.875018427444851,
1.),(1.,0.874619707139394,1.)))
REPRESENTATION_ITEM('')
SURFACE()
);
#3425=(
BOUNDED_SURFACE()
B_SPLINE_SURFACE(3,2,((#244196,#244197,#244198),(#244199,#244200,#244201),
(#244202,#244203,#244204),(#244205,#244206,#244207)),.UNSPECIFIED.,.F.,
 .F.,.F.)
B_SPLINE_SURFACE_WITH_KNOTS((4,4),(3,3),(5.96311194867027E-19,0.000511815072430393),
(0.,1.00105598365887),.UNSPECIFIED.)
GEOMETRIC_REPRESENTATION_ITEM()
RATIONAL_B_SPLINE_SURFACE(((1.,0.706797490733686,1.00061923411705),(1.,
0.706182062146616,1.00062053388211),(1.,0.70558406276894,1.00062179683726),
(1.,0.705266224770434,1.00062246810072)))
REPRESENTATION_ITEM('')
SURFACE()
);
#3426=(
BOUNDED_SURFACE()
B_SPLINE_SURFACE(3,2,((#244213,#244214,#244215),(#244216,#244217,#244218),
(#244219,#244220,#244221),(#244222,#244223,#244224),(#244225,#244226,#244227),
(#244228,#244229,#244230)),.UNSPECIFIED.,.F.,.F.,.F.)
B_SPLINE_SURFACE_WITH_KNOTS((4,2,4),(3,3),(0.,0.000257652232350883,0.000515304464701765),
(0.,1.),.UNSPECIFIED.)
GEOMETRIC_REPRESENTATION_ITEM()
RATIONAL_B_SPLINE_SURFACE(((1.,0.874619707139395,1.),(1.,0.874861180431021,
1.),(1.,0.855455725920468,1.),(1.,0.794699358955673,1.),(1.,0.753768977788341,
1.),(1.,0.708712527163671,1.)))
REPRESENTATION_ITEM('')
SURFACE()
);
#3427=(
BOUNDED_SURFACE()
B_SPLINE_SURFACE(3,2,((#244236,#244237,#244238),(#244239,#244240,#244241),
(#244242,#244243,#244244),(#244245,#244246,#244247)),.UNSPECIFIED.,.F.,
 .F.,.F.)
B_SPLINE_SURFACE_WITH_KNOTS((4,4),(3,3),(0.,0.000397394373651922),(0.,1.),
 .UNSPECIFIED.)
GEOMETRIC_REPRESENTATION_ITEM()
RATIONAL_B_SPLINE_SURFACE(((1.,0.707106781186548,1.),(1.,0.707752587915897,
1.),(1.,0.708377654540704,1.),(1.,0.708689770883339,1.)))
REPRESENTATION_ITEM('')
SURFACE()
);
#3428=(
BOUNDED_SURFACE()
B_SPLINE_SURFACE(3,2,((#244249,#244250,#244251),(#244252,#244253,#244254),
(#244255,#244256,#244257),(#244258,#244259,#244260)),.UNSPECIFIED.,.F.,
 .F.,.F.)
B_SPLINE_SURFACE_WITH_KNOTS((4,4),(3,3),(0.,0.000511815456479789),(0.,1.00105873159825),
 .UNSPECIFIED.)
GEOMETRIC_REPRESENTATION_ITEM()
RATIONAL_B_SPLINE_SURFACE(((1.,0.708394529056854,1.00061746385262),(1.,
0.708058564167349,1.00061817524591),(1.,0.707430835372582,1.00061950443853),
(1.,0.706796685880876,1.00062084722674)))
REPRESENTATION_ITEM('')
SURFACE()
);
#3429=(
BOUNDED_SURFACE()
B_SPLINE_SURFACE(3,2,((#244266,#244267,#244268),(#244269,#244270,#244271),
(#244272,#244273,#244274),(#244275,#244276,#244277)),.UNSPECIFIED.,.F.,
 .F.,.F.)
B_SPLINE_SURFACE_WITH_KNOTS((4,4),(3,3),(0.,0.000397394465448316),(0.,1.),
 .UNSPECIFIED.)
GEOMETRIC_REPRESENTATION_ITEM()
RATIONAL_B_SPLINE_SURFACE(((1.,0.705498956110759,1.),(1.,0.705821764811766,
1.),(1.,0.706461952521144,1.),(1.,0.707106781186546,1.)))
REPRESENTATION_ITEM('')
SURFACE()
);
#3430=(
BOUNDED_SURFACE()
B_SPLINE_SURFACE(3,2,((#244283,#244284,#244285),(#244286,#244287,#244288),
(#244289,#244290,#244291),(#244292,#244293,#244294)),.UNSPECIFIED.,.F.,
 .F.,.F.)
B_SPLINE_SURFACE_WITH_KNOTS((4,4),(3,3),(0.,0.000397394410828743),(0.,1.),
 .UNSPECIFIED.)
GEOMETRIC_REPRESENTATION_ITEM()
RATIONAL_B_SPLINE_SURFACE(((1.,0.708689770883332,1.),(1.,0.70837644003449,
1.),(1.,0.707750498698407,1.),(1.,0.707106781186551,1.)))
REPRESENTATION_ITEM('')
SURFACE()
);
#3431=(
BOUNDED_SURFACE()
B_SPLINE_SURFACE(3,2,((#244300,#244301,#244302),(#244303,#244304,#244305),
(#244306,#244307,#244308),(#244309,#244310,#244311)),.UNSPECIFIED.,.F.,
 .F.,.F.)
B_SPLINE_SURFACE_WITH_KNOTS((4,4),(3,3),(0.,0.000511815090126169),(0.,1.00105592270137),
 .UNSPECIFIED.)
GEOMETRIC_REPRESENTATION_ITEM()
RATIONAL_B_SPLINE_SURFACE(((1.,0.705266242717729,1.00062243213035),(1.,
0.70558408590941,1.00062176089466),(1.,0.706182089450716,1.00062049800363),
(1.,0.706797508587726,1.00061919833356)))
REPRESENTATION_ITEM('')
SURFACE()
);
#3432=(
BOUNDED_SURFACE()
B_SPLINE_SURFACE(3,2,((#244313,#244314,#244315),(#244316,#244317,#244318),
(#244319,#244320,#244321),(#244322,#244323,#244324)),.UNSPECIFIED.,.F.,
 .F.,.F.)
B_SPLINE_SURFACE_WITH_KNOTS((4,4),(3,3),(0.,0.00039739442808661),(0.,1.),
 .UNSPECIFIED.)
GEOMETRIC_REPRESENTATION_ITEM()
RATIONAL_B_SPLINE_SURFACE(((1.,0.707106781186552,1.),(1.,0.70645984675909,
1.),(1.,0.705820510737272,1.),(1.,0.705498956110746,1.)))
REPRESENTATION_ITEM('')
SURFACE()
);
#3433=(
BOUNDED_SURFACE()
B_SPLINE_SURFACE(3,2,((#244330,#244331,#244332),(#244333,#244334,#244335),
(#244336,#244337,#244338),(#244339,#244340,#244341),(#244342,#244343,#244344),
(#244345,#244346,#244347)),.UNSPECIFIED.,.F.,.F.,.F.)
B_SPLINE_SURFACE_WITH_KNOTS((4,2,4),(3,3),(0.,0.000257953807872836,0.000515907615745672),
(0.,1.),.UNSPECIFIED.)
GEOMETRIC_REPRESENTATION_ITEM()
RATIONAL_B_SPLINE_SURFACE(((1.,0.874619707139391,1.),(1.,0.874834349679291,
1.),(1.,0.854686104157408,1.),(1.,0.792476597915517,1.),(1.,0.750887854594871,
1.),(1.,0.705585838031449,1.)))
REPRESENTATION_ITEM('')
SURFACE()
);
#3434=(
BOUNDED_SURFACE()
B_SPLINE_SURFACE(3,2,((#244353,#244354,#244355),(#244356,#244357,#244358),
(#244359,#244360,#244361),(#244362,#244363,#244364)),.UNSPECIFIED.,.F.,
 .F.,.F.)
B_SPLINE_SURFACE_WITH_KNOTS((4,4),(3,3),(0.,0.00051181543769915),(0.,1.00105881331569),
 .UNSPECIFIED.)
GEOMETRIC_REPRESENTATION_ITEM()
RATIONAL_B_SPLINE_SURFACE(((1.,0.706796661946389,1.00062089519707),(1.,
0.707430821225278,1.00061955228449),(1.,0.708058545830776,1.00061822299815),
(1.,0.708394505252776,1.00061751156153)))
REPRESENTATION_ITEM('')
SURFACE()
);
#3435=(
BOUNDED_SURFACE()
B_SPLINE_SURFACE(3,2,((#244366,#244367,#244368),(#244369,#244370,#244371),
(#244372,#244373,#244374),(#244375,#244376,#244377),(#244378,#244379,#244380),
(#244381,#244382,#244383)),.UNSPECIFIED.,.F.,.F.,.F.)
B_SPLINE_SURFACE_WITH_KNOTS((4,2,4),(3,3),(0.,0.000256915317531256,0.000513830635062512),
(0.,1.),.UNSPECIFIED.)
GEOMETRIC_REPRESENTATION_ITEM()
RATIONAL_B_SPLINE_SURFACE(((1.,0.705585838031447,1.),(1.,0.750902433541732,
1.),(1.,0.792329530083833,1.),(1.,0.854288401592882,1.),(1.,0.874998031126119,
1.),(1.,0.874619707139395,1.)))
REPRESENTATION_ITEM('')
SURFACE()
);
#3436=(
BOUNDED_SURFACE()
B_SPLINE_SURFACE(3,2,((#244389,#244390,#244391),(#244392,#244393,#244394),
(#244395,#244396,#244397),(#244398,#244399,#244400),(#244401,#244402,#244403),
(#244404,#244405,#244406)),.UNSPECIFIED.,.F.,.F.,.F.)
B_SPLINE_SURFACE_WITH_KNOTS((4,2,4),(3,3),(-2.5207700510288E-18,0.000256592814262155,
0.000513185628524313),(0.,1.),.UNSPECIFIED.)
GEOMETRIC_REPRESENTATION_ITEM()
RATIONAL_B_SPLINE_SURFACE(((1.,0.70871252716366,1.),(1.,0.753780902613132,
1.),(1.,0.794538995769815,1.),(1.,0.855070770330497,1.),(1.,0.875018427445787,
1.),(1.,0.874619707139398,1.)))
REPRESENTATION_ITEM('')
SURFACE()
);
#3437=(
BOUNDED_SURFACE()
B_SPLINE_SURFACE(3,2,((#244408,#244409,#244410),(#244411,#244412,#244413),
(#244414,#244415,#244416),(#244417,#244418,#244419)),.UNSPECIFIED.,.F.,
 .F.,.F.)
B_SPLINE_SURFACE_WITH_KNOTS((4,4),(3,3),(5.96311194867027E-19,0.000511815072430402),
(0.,1.00105598365777),.UNSPECIFIED.)
GEOMETRIC_REPRESENTATION_ITEM()
RATIONAL_B_SPLINE_SURFACE(((1.,0.706797490734009,1.0006192341164),(1.,0.706182062146925,
1.00062053388146),(1.,0.705584062769296,1.0006217968366),(1.,0.705266224770765,
1.00062246810007)))
REPRESENTATION_ITEM('')
SURFACE()
);
#3438=(
BOUNDED_SURFACE()
B_SPLINE_SURFACE(3,2,((#244425,#244426,#244427),(#244428,#244429,#244430),
(#244431,#244432,#244433),(#244434,#244435,#244436),(#244437,#244438,#244439),
(#244440,#244441,#244442)),.UNSPECIFIED.,.F.,.F.,.F.)
B_SPLINE_SURFACE_WITH_KNOTS((4,2,4),(3,3),(0.,0.00025765223235088,0.00051530446470176),
(0.,1.),.UNSPECIFIED.)
GEOMETRIC_REPRESENTATION_ITEM()
RATIONAL_B_SPLINE_SURFACE(((1.,0.874619707139393,1.),(1.,0.874861180430485,
1.),(1.,0.8554557259212,1.),(1.,0.794699358954937,1.),(1.,0.753768977788887,
1.),(1.,0.708712527163683,1.)))
REPRESENTATION_ITEM('')
SURFACE()
);
#3439=(
BOUNDED_SURFACE()
B_SPLINE_SURFACE(3,2,((#244448,#244449,#244450),(#244451,#244452,#244453),
(#244454,#244455,#244456),(#244457,#244458,#244459)),.UNSPECIFIED.,.F.,
 .F.,.F.)
B_SPLINE_SURFACE_WITH_KNOTS((4,4),(3,3),(0.,0.000397394373651921),(0.,1.),
 .UNSPECIFIED.)
GEOMETRIC_REPRESENTATION_ITEM()
RATIONAL_B_SPLINE_SURFACE(((1.,0.707106781186548,1.),(1.,0.70775258791588,
1.),(1.,0.708377654540694,1.),(1.,0.70868977088333,1.)))
REPRESENTATION_ITEM('')
SURFACE()
);
#3440=(
BOUNDED_SURFACE()
B_SPLINE_SURFACE(3,2,((#244461,#244462,#244463),(#244464,#244465,#244466),
(#244467,#244468,#244469),(#244470,#244471,#244472)),.UNSPECIFIED.,.F.,
 .F.,.F.)
B_SPLINE_SURFACE_WITH_KNOTS((4,4),(3,3),(0.,0.000511815456479791),(0.,1.00105873159742),
 .UNSPECIFIED.)
GEOMETRIC_REPRESENTATION_ITEM()
RATIONAL_B_SPLINE_SURFACE(((1.,0.708394529057083,1.00061746385214),(1.,
0.708058564167601,1.00061817524542),(1.,0.707430835372811,1.00061950443804),
(1.,0.70679668588112,1.00062084722625)))
REPRESENTATION_ITEM('')
SURFACE()
);
#3441=(
BOUNDED_SURFACE()
B_SPLINE_SURFACE(3,2,((#244478,#244479,#244480),(#244481,#244482,#244483),
(#244484,#244485,#244486),(#244487,#244488,#244489)),.UNSPECIFIED.,.F.,
 .F.,.F.)
B_SPLINE_SURFACE_WITH_KNOTS((4,4),(3,3),(0.,0.000397394465448304),(0.,1.),
 .UNSPECIFIED.)
GEOMETRIC_REPRESENTATION_ITEM()
RATIONAL_B_SPLINE_SURFACE(((1.,0.705498956110762,1.),(1.,0.705821764811753,
1.),(1.,0.706461952521157,1.),(1.,0.707106781186548,1.)))
REPRESENTATION_ITEM('')
SURFACE()
);
#3442=(
BOUNDED_SURFACE()
B_SPLINE_SURFACE(3,2,((#244495,#244496,#244497),(#244498,#244499,#244500),
(#244501,#244502,#244503),(#244504,#244505,#244506)),.UNSPECIFIED.,.F.,
 .F.,.F.)
B_SPLINE_SURFACE_WITH_KNOTS((4,4),(3,3),(0.,0.000397394410828741),(0.,1.),
 .UNSPECIFIED.)
GEOMETRIC_REPRESENTATION_ITEM()
RATIONAL_B_SPLINE_SURFACE(((1.,0.708689770883328,1.),(1.,0.708376440034484,
1.),(1.,0.7077504986984,1.),(1.,0.707106781186561,1.)))
REPRESENTATION_ITEM('')
SURFACE()
);
#3443=(
BOUNDED_SURFACE()
B_SPLINE_SURFACE(3,2,((#244512,#244513,#244514),(#244515,#244516,#244517),
(#244518,#244519,#244520),(#244521,#244522,#244523)),.UNSPECIFIED.,.F.,
 .F.,.F.)
B_SPLINE_SURFACE_WITH_KNOTS((4,4),(3,3),(0.,0.000511815090126166),(0.,1.00105592270446),
 .UNSPECIFIED.)
GEOMETRIC_REPRESENTATION_ITEM()
RATIONAL_B_SPLINE_SURFACE(((1.,0.705266242716819,1.00062243213217),(1.,
0.705584085908485,1.00062176089648),(1.,0.706182089449831,1.00062049800545),
(1.,0.706797508586823,1.00061919833537)))
REPRESENTATION_ITEM('')
SURFACE()
);
#3444=(
BOUNDED_SURFACE()
B_SPLINE_SURFACE(3,2,((#244525,#244526,#244527),(#244528,#244529,#244530),
(#244531,#244532,#244533),(#244534,#244535,#244536)),.UNSPECIFIED.,.F.,
 .F.,.F.)
B_SPLINE_SURFACE_WITH_KNOTS((4,4),(3,3),(5.6920614055489E-19,0.000397394428086632),
(0.,1.),.UNSPECIFIED.)
GEOMETRIC_REPRESENTATION_ITEM()
RATIONAL_B_SPLINE_SURFACE(((1.,0.707106781186555,1.),(1.,0.706459846759096,
1.),(1.,0.705820510737272,1.),(1.,0.705498956110754,1.)))
REPRESENTATION_ITEM('')
SURFACE()
);
#3445=(
BOUNDED_SURFACE()
B_SPLINE_SURFACE(3,2,((#244542,#244543,#244544),(#244545,#244546,#244547),
(#244548,#244549,#244550),(#244551,#244552,#244553),(#244554,#244555,#244556),
(#244557,#244558,#244559)),.UNSPECIFIED.,.F.,.F.,.F.)
B_SPLINE_SURFACE_WITH_KNOTS((4,2,4),(3,3),(0.,0.000257953807872845,0.00051590761574569),
(0.,1.),.UNSPECIFIED.)
GEOMETRIC_REPRESENTATION_ITEM()
RATIONAL_B_SPLINE_SURFACE(((1.,0.874619707139396,1.),(1.,0.874834349679282,
1.),(1.,0.854686104157417,1.),(1.,0.792476597915543,1.),(1.,0.750887854594793,
1.),(1.,0.705585838031461,1.)))
REPRESENTATION_ITEM('')
SURFACE()
);
#3446=(
BOUNDED_SURFACE()
B_SPLINE_SURFACE(3,2,((#244565,#244566,#244567),(#244568,#244569,#244570),
(#244571,#244572,#244573),(#244574,#244575,#244576)),.UNSPECIFIED.,.F.,
 .F.,.F.)
B_SPLINE_SURFACE_WITH_KNOTS((4,4),(3,3),(0.,0.000511815437699145),(0.,1.00105881331729),
 .UNSPECIFIED.)
GEOMETRIC_REPRESENTATION_ITEM()
RATIONAL_B_SPLINE_SURFACE(((1.,0.706796661945924,1.00062089519801),(1.,
0.707430821224786,1.00061955228543),(1.,0.708058545830317,1.00061822299909),
(1.,0.708394505252299,1.00061751156247)))
REPRESENTATION_ITEM('')
SURFACE()
);
#3447=(
BOUNDED_SURFACE()
B_SPLINE_SURFACE(3,2,((#244578,#244579,#244580),(#244581,#244582,#244583),
(#244584,#244585,#244586),(#244587,#244588,#244589),(#244590,#244591,#244592),
(#244593,#244594,#244595)),.UNSPECIFIED.,.F.,.F.,.F.)
B_SPLINE_SURFACE_WITH_KNOTS((4,2,4),(3,3),(0.,0.00025691531753127,0.00051383063506254),
(0.,1.),.UNSPECIFIED.)
GEOMETRIC_REPRESENTATION_ITEM()
RATIONAL_B_SPLINE_SURFACE(((1.,0.705585838031444,1.),(1.,0.75090243354346,
1.),(1.,0.792329530081589,1.),(1.,0.854288401595151,1.),(1.,0.874998031124432,
1.),(1.,0.87461970713941,1.)))
REPRESENTATION_ITEM('')
SURFACE()
);
#3448=(
BOUNDED_SURFACE()
B_SPLINE_SURFACE(3,2,((#244601,#244602,#244603),(#244604,#244605,#244606),
(#244607,#244608,#244609),(#244610,#244611,#244612),(#244613,#244614,#244615),
(#244616,#244617,#244618)),.UNSPECIFIED.,.F.,.F.,.F.)
B_SPLINE_SURFACE_WITH_KNOTS((4,2,4),(3,3),(-3.95733792957209E-18,0.000256592814262154,
0.000513185628524312),(0.,1.),.UNSPECIFIED.)
GEOMETRIC_REPRESENTATION_ITEM()
RATIONAL_B_SPLINE_SURFACE(((1.,0.708712527163665,1.),(1.,0.753780902613942,
1.),(1.,0.794538995768714,1.),(1.,0.855070770331582,1.),(1.,0.875018427444968,
1.),(1.,0.874619707139392,1.)))
REPRESENTATION_ITEM('')
SURFACE()
);
#3449=(
BOUNDED_SURFACE()
B_SPLINE_SURFACE(3,2,((#244620,#244621,#244622),(#244623,#244624,#244625),
(#244626,#244627,#244628),(#244629,#244630,#244631)),.UNSPECIFIED.,.F.,
 .F.,.F.)
B_SPLINE_SURFACE_WITH_KNOTS((4,4),(3,3),(5.6920614055489E-19,0.000511815072430398),
(0.,1.00105598366039),.UNSPECIFIED.)
GEOMETRIC_REPRESENTATION_ITEM()
RATIONAL_B_SPLINE_SURFACE(((1.,0.706797490733239,1.00061923411794),(1.,
0.706182062146141,1.00062053388301),(1.,0.705584062768533,1.00062179683815),
(1.,0.70526622476999,1.00062246810162)))
REPRESENTATION_ITEM('')
SURFACE()
);
#3450=(
BOUNDED_SURFACE()
B_SPLINE_SURFACE(3,2,((#244637,#244638,#244639),(#244640,#244641,#244642),
(#244643,#244644,#244645),(#244646,#244647,#244648),(#244649,#244650,#244651),
(#244652,#244653,#244654)),.UNSPECIFIED.,.F.,.F.,.F.)
B_SPLINE_SURFACE_WITH_KNOTS((4,2,4),(3,3),(-3.42878937048541E-18,0.000257652232350883,
0.000515304464701769),(0.,1.),.UNSPECIFIED.)
GEOMETRIC_REPRESENTATION_ITEM()
RATIONAL_B_SPLINE_SURFACE(((1.,0.874619707139372,1.),(1.,0.874861180430602,
1.),(1.,0.855455725920989,1.),(1.,0.794699358955127,1.),(1.,0.753768977788718,
1.),(1.,0.70871252716366,1.)))
REPRESENTATION_ITEM('')
SURFACE()
);
#3451=(
BOUNDED_SURFACE()
B_SPLINE_SURFACE(3,2,((#244660,#244661,#244662),(#244663,#244664,#244665),
(#244666,#244667,#244668),(#244669,#244670,#244671)),.UNSPECIFIED.,.F.,
 .F.,.F.)
B_SPLINE_SURFACE_WITH_KNOTS((4,4),(3,3),(0.,0.000397394373651921),(0.,1.),
 .UNSPECIFIED.)
GEOMETRIC_REPRESENTATION_ITEM()
RATIONAL_B_SPLINE_SURFACE(((1.,0.70710678118654,1.),(1.,0.707752587915911,
1.),(1.,0.70837765454067,1.),(1.,0.708689770883334,1.)))
REPRESENTATION_ITEM('')
SURFACE()
);
#3452=(
BOUNDED_SURFACE()
B_SPLINE_SURFACE(3,2,((#244673,#244674,#244675),(#244676,#244677,#244678),
(#244679,#244680,#244681),(#244682,#244683,#244684)),.UNSPECIFIED.,.F.,
 .F.,.F.)
B_SPLINE_SURFACE_WITH_KNOTS((4,4),(3,3),(-1.59919820441612E-18,0.000511815456479788),
(0.,1.00105873159859),.UNSPECIFIED.)
GEOMETRIC_REPRESENTATION_ITEM()
RATIONAL_B_SPLINE_SURFACE(((1.,0.708394529056712,1.00061746385282),(1.,
0.708058564167312,1.00061817524611),(1.,0.70743083537244,1.00061950443873),
(1.,0.70679668588077,1.00062084722694)))
REPRESENTATION_ITEM('')
SURFACE()
);
#3453=(
BOUNDED_SURFACE()
B_SPLINE_SURFACE(3,2,((#244690,#244691,#244692),(#244693,#244694,#244695),
(#244696,#244697,#244698),(#244699,#244700,#244701)),.UNSPECIFIED.,.F.,
 .F.,.F.)
B_SPLINE_SURFACE_WITH_KNOTS((4,4),(3,3),(0.,0.000397394465448327),(0.,1.),
 .UNSPECIFIED.)
GEOMETRIC_REPRESENTATION_ITEM()
RATIONAL_B_SPLINE_SURFACE(((1.,0.705498956110748,1.),(1.,0.705821764811772,
1.),(1.,0.706461952521144,1.),(1.,0.707106781186546,1.)))
REPRESENTATION_ITEM('')
SURFACE()
);
#3454=(
BOUNDED_SURFACE()
B_SPLINE_SURFACE(3,2,((#244707,#244708,#244709),(#244710,#244711,#244712),
(#244713,#244714,#244715),(#244716,#244717,#244718)),.UNSPECIFIED.,.F.,
 .F.,.F.)
B_SPLINE_SURFACE_WITH_KNOTS((4,4),(3,3),(0.,0.000397394410828723),(0.,1.),
 .UNSPECIFIED.)
GEOMETRIC_REPRESENTATION_ITEM()
RATIONAL_B_SPLINE_SURFACE(((1.,0.708689770883336,1.),(1.,0.70837644003447,
1.),(1.,0.707750498698429,1.),(1.,0.707106781186541,1.)))
REPRESENTATION_ITEM('')
SURFACE()
);
#3455=(
BOUNDED_SURFACE()
B_SPLINE_SURFACE(3,2,((#244724,#244725,#244726),(#244727,#244728,#244729),
(#244730,#244731,#244732),(#244733,#244734,#244735)),.UNSPECIFIED.,.F.,
 .F.,.F.)
B_SPLINE_SURFACE_WITH_KNOTS((4,4),(3,3),(-4.01154803819637E-18,0.000511815090126176),
(0.,1.00105592270494),.UNSPECIFIED.)
GEOMETRIC_REPRESENTATION_ITEM()
RATIONAL_B_SPLINE_SURFACE(((1.,0.705266242716679,1.00062243213246),(1.,
0.705584085908372,1.00062176089677),(1.,0.706182089449679,1.00062049800574),
(1.,0.70679750858668,1.00061919833566)))
REPRESENTATION_ITEM('')
SURFACE()
);
#3456=(
BOUNDED_SURFACE()
B_SPLINE_SURFACE(3,2,((#244737,#244738,#244739),(#244740,#244741,#244742),
(#244743,#244744,#244745),(#244746,#244747,#244748)),.UNSPECIFIED.,.F.,
 .F.,.F.)
B_SPLINE_SURFACE_WITH_KNOTS((4,4),(3,3),(0.,0.000397394428086601),(0.,1.),
 .UNSPECIFIED.)
GEOMETRIC_REPRESENTATION_ITEM()
RATIONAL_B_SPLINE_SURFACE(((1.,0.707106781186548,1.),(1.,0.706459846759071,
1.),(1.,0.705820510737329,1.),(1.,0.70549895611073,1.)))
REPRESENTATION_ITEM('')
SURFACE()
);
#3457=(
BOUNDED_SURFACE()
B_SPLINE_SURFACE(3,2,((#244754,#244755,#244756),(#244757,#244758,#244759),
(#244760,#244761,#244762),(#244763,#244764,#244765),(#244766,#244767,#244768),
(#244769,#244770,#244771)),.UNSPECIFIED.,.F.,.F.,.F.)
B_SPLINE_SURFACE_WITH_KNOTS((4,2,4),(3,3),(0.,0.000257953807872844,0.000515907615745688),
(0.,1.),.UNSPECIFIED.)
GEOMETRIC_REPRESENTATION_ITEM()
RATIONAL_B_SPLINE_SURFACE(((1.,0.874619707139391,1.),(1.,0.874834349679489,
1.),(1.,0.854686104157156,1.),(1.,0.792476597915762,1.),(1.,0.750887854594684,
1.),(1.,0.705585838031417,1.)))
REPRESENTATION_ITEM('')
SURFACE()
);
#3458=(
BOUNDED_SURFACE()
B_SPLINE_SURFACE(3,2,((#244777,#244778,#244779),(#244780,#244781,#244782),
(#244783,#244784,#244785),(#244786,#244787,#244788)),.UNSPECIFIED.,.F.,
 .F.,.F.)
B_SPLINE_SURFACE_WITH_KNOTS((4,4),(3,3),(-5.6920614055489E-19,0.00051181543769916),
(0.,1.00105881331573),.UNSPECIFIED.)
GEOMETRIC_REPRESENTATION_ITEM()
RATIONAL_B_SPLINE_SURFACE(((1.,0.706796661946382,1.0006208951971),(1.,0.707430821225235,
1.00061955228452),(1.,0.708058545830781,1.00061822299818),(1.,0.708394505252767,
1.00061751156156)))
REPRESENTATION_ITEM('')
SURFACE()
);
#3459=(
BOUNDED_SURFACE()
B_SPLINE_SURFACE(3,2,((#244790,#244791,#244792),(#244793,#244794,#244795),
(#244796,#244797,#244798),(#244799,#244800,#244801),(#244802,#244803,#244804),
(#244805,#244806,#244807)),.UNSPECIFIED.,.F.,.F.,.F.)
B_SPLINE_SURFACE_WITH_KNOTS((4,2,4),(3,3),(-3.52365706057789E-19,0.000256915317531259,
0.000513830635062519),(0.,1.),.UNSPECIFIED.)
GEOMETRIC_REPRESENTATION_ITEM()
RATIONAL_B_SPLINE_SURFACE(((1.,0.705585838031437,1.),(1.,0.750902433542628,
1.),(1.,0.792329530082712,1.),(1.,0.854288401594017,1.),(1.,0.874998031125283,
1.),(1.,0.87461970713941,1.)))
REPRESENTATION_ITEM('')
SURFACE()
);
#3460=(
BOUNDED_SURFACE()
B_SPLINE_SURFACE(3,2,((#244813,#244814,#244815),(#244816,#244817,#244818),
(#244819,#244820,#244821),(#244822,#244823,#244824),(#244825,#244826,#244827),
(#244828,#244829,#244830)),.UNSPECIFIED.,.F.,.F.,.F.)
B_SPLINE_SURFACE_WITH_KNOTS((4,2,4),(3,3),(0.,0.000256592814262159,0.000513185628524318),
(0.,1.),.UNSPECIFIED.)
GEOMETRIC_REPRESENTATION_ITEM()
RATIONAL_B_SPLINE_SURFACE(((1.,0.708712527163661,1.),(1.,0.753780902613338,
1.),(1.,0.794538995769515,1.),(1.,0.855070770330818,1.),(1.,0.875018427445545,
1.),(1.,0.874619707139392,1.)))
REPRESENTATION_ITEM('')
SURFACE()
);
#3461=(
BOUNDED_SURFACE()
B_SPLINE_SURFACE(3,2,((#244832,#244833,#244834),(#244835,#244836,#244837),
(#244838,#244839,#244840),(#244841,#244842,#244843)),.UNSPECIFIED.,.F.,
 .F.,.F.)
B_SPLINE_SURFACE_WITH_KNOTS((4,4),(3,3),(-2.71050543121376E-20,0.000511815072430398),
(0.,1.00105598365999),.UNSPECIFIED.)
GEOMETRIC_REPRESENTATION_ITEM()
RATIONAL_B_SPLINE_SURFACE(((1.,0.706797490733357,1.00061923411771),(1.,
0.706182062146283,1.00062053388277),(1.,0.705584062768626,1.00062179683791),
(1.,0.705266224770118,1.00062246810138)))
REPRESENTATION_ITEM('')
SURFACE()
);
#3462=(
BOUNDED_SURFACE()
B_SPLINE_SURFACE(3,2,((#244849,#244850,#244851),(#244852,#244853,#244854),
(#244855,#244856,#244857),(#244858,#244859,#244860),(#244861,#244862,#244863),
(#244864,#244865,#244866)),.UNSPECIFIED.,.F.,.F.,.F.)
B_SPLINE_SURFACE_WITH_KNOTS((4,2,4),(3,3),(0.,0.000257652232350886,0.000515304464701772),
(0.,1.),.UNSPECIFIED.)
GEOMETRIC_REPRESENTATION_ITEM()
RATIONAL_B_SPLINE_SURFACE(((1.,0.874619707139399,1.),(1.,0.874861180430627,
1.),(1.,0.855455725920946,1.),(1.,0.794699358955181,1.),(1.,0.753768977788717,
1.),(1.,0.70871252716364,1.)))
REPRESENTATION_ITEM('')
SURFACE()
);
#3463=(
BOUNDED_SURFACE()
B_SPLINE_SURFACE(3,2,((#244872,#244873,#244874),(#244875,#244876,#244877),
(#244878,#244879,#244880),(#244881,#244882,#244883)),.UNSPECIFIED.,.F.,
 .F.,.F.)
B_SPLINE_SURFACE_WITH_KNOTS((4,4),(3,3),(-6.50521303491303E-19,0.000397394373651923),
(0.,1.),.UNSPECIFIED.)
GEOMETRIC_REPRESENTATION_ITEM()
RATIONAL_B_SPLINE_SURFACE(((1.,0.707106781186546,1.),(1.,0.707752587915898,
1.),(1.,0.708377654540671,1.),(1.,0.708689770883336,1.)))
REPRESENTATION_ITEM('')
SURFACE()
);
#3464=(
BOUNDED_SURFACE()
B_SPLINE_SURFACE(3,2,((#244885,#244886,#244887),(#244888,#244889,#244890),
(#244891,#244892,#244893),(#244894,#244895,#244896)),.UNSPECIFIED.,.F.,
 .F.,.F.)
B_SPLINE_SURFACE_WITH_KNOTS((4,4),(3,3),(0.,0.000511815456479791),(0.,1.00105873160122),
 .UNSPECIFIED.)
GEOMETRIC_REPRESENTATION_ITEM()
RATIONAL_B_SPLINE_SURFACE(((1.,0.708394529055968,1.00061746385436),(1.,
0.708058564166503,1.00061817524765),(1.,0.707430835371682,1.00061950444027),
(1.,0.706796685880003,1.00062084722849)))
REPRESENTATION_ITEM('')
SURFACE()
);
#3465=(
BOUNDED_SURFACE()
B_SPLINE_SURFACE(3,2,((#244902,#244903,#244904),(#244905,#244906,#244907),
(#244908,#244909,#244910),(#244911,#244912,#244913)),.UNSPECIFIED.,.F.,
 .F.,.F.)
B_SPLINE_SURFACE_WITH_KNOTS((4,4),(3,3),(0.,0.0003973944654483),(0.,1.),
 .UNSPECIFIED.)
GEOMETRIC_REPRESENTATION_ITEM()
RATIONAL_B_SPLINE_SURFACE(((1.,0.705498956110742,1.),(1.,0.70582176481179,
1.),(1.,0.70646195252114,1.),(1.,0.707106781186547,1.)))
REPRESENTATION_ITEM('')
SURFACE()
);
#3466=(
BOUNDED_SURFACE()
B_SPLINE_SURFACE(3,2,((#244919,#244920,#244921),(#244922,#244923,#244924),
(#244925,#244926,#244927),(#244928,#244929,#244930)),.UNSPECIFIED.,.F.,
 .F.,.F.)
B_SPLINE_SURFACE_WITH_KNOTS((4,4),(3,3),(0.,0.000397394410828726),(0.,1.),
 .UNSPECIFIED.)
GEOMETRIC_REPRESENTATION_ITEM()
RATIONAL_B_SPLINE_SURFACE(((1.,0.708689770883339,1.),(1.,0.708376440034475,
1.),(1.,0.707750498698421,1.),(1.,0.707106781186549,1.)))
REPRESENTATION_ITEM('')
SURFACE()
);
#3467=(
BOUNDED_SURFACE()
B_SPLINE_SURFACE(3,2,((#244936,#244937,#244938),(#244939,#244940,#244941),
(#244942,#244943,#244944),(#244945,#244946,#244947)),.UNSPECIFIED.,.F.,
 .F.,.F.)
B_SPLINE_SURFACE_WITH_KNOTS((4,4),(3,3),(-3.22550146314438E-18,0.00051181509012618),
(0.,1.00105592270442),.UNSPECIFIED.)
GEOMETRIC_REPRESENTATION_ITEM()
RATIONAL_B_SPLINE_SURFACE(((1.,0.705266242716829,1.00062243213215),(1.,
0.70558408590849,1.00062176089647),(1.,0.706182089449834,1.00062049800543),
(1.,0.706797508586832,1.00061919833535)))
REPRESENTATION_ITEM('')
SURFACE()
);
#3468=(
BOUNDED_SURFACE()
B_SPLINE_SURFACE(3,2,((#244949,#244950,#244951),(#244952,#244953,#244954),
(#244955,#244956,#244957),(#244958,#244959,#244960)),.UNSPECIFIED.,.F.,
 .F.,.F.)
B_SPLINE_SURFACE_WITH_KNOTS((4,4),(3,3),(0.,0.00039739442808661),(0.,1.),
 .UNSPECIFIED.)
GEOMETRIC_REPRESENTATION_ITEM()
RATIONAL_B_SPLINE_SURFACE(((1.,0.70710678118654,1.),(1.,0.706459846759122,
1.),(1.,0.705820510737254,1.),(1.,0.705498956110749,1.)))
REPRESENTATION_ITEM('')
SURFACE()
);
#3469=(
BOUNDED_SURFACE()
B_SPLINE_SURFACE(3,2,((#244966,#244967,#244968),(#244969,#244970,#244971),
(#244972,#244973,#244974),(#244975,#244976,#244977),(#244978,#244979,#244980),
(#244981,#244982,#244983)),.UNSPECIFIED.,.F.,.F.,.F.)
B_SPLINE_SURFACE_WITH_KNOTS((4,2,4),(3,3),(0.,0.000257953807872843,0.000515907615745687),
(0.,1.),.UNSPECIFIED.)
GEOMETRIC_REPRESENTATION_ITEM()
RATIONAL_B_SPLINE_SURFACE(((1.,0.874619707139395,1.),(1.,0.874834349679314,
1.),(1.,0.854686104157372,1.),(1.,0.792476597915575,1.),(1.,0.750887854594771,
1.),(1.,0.705585838031435,1.)))
REPRESENTATION_ITEM('')
SURFACE()
);
#3470=(
BOUNDED_SURFACE()
B_SPLINE_SURFACE(3,2,((#244989,#244990,#244991),(#244992,#244993,#244994),
(#244995,#244996,#244997),(#244998,#244999,#245000)),.UNSPECIFIED.,.F.,
 .F.,.F.)
B_SPLINE_SURFACE_WITH_KNOTS((4,4),(3,3),(-5.6920614055489E-19,0.000511815437699148),
(0.,1.00105881331991),.UNSPECIFIED.)
GEOMETRIC_REPRESENTATION_ITEM()
RATIONAL_B_SPLINE_SURFACE(((1.,0.706796661945167,1.00062089519955),(1.,
0.707430821224023,1.00061955228697),(1.,0.70805854582955,1.00061822300062),
(1.,0.708394505251536,1.000617511564)))
REPRESENTATION_ITEM('')
SURFACE()
);
#3471=(
BOUNDED_SURFACE()
B_SPLINE_SURFACE(3,2,((#245002,#245003,#245004),(#245005,#245006,#245007),
(#245008,#245009,#245010),(#245011,#245012,#245013),(#245014,#245015,#245016),
(#245017,#245018,#245019)),.UNSPECIFIED.,.F.,.F.,.F.)
B_SPLINE_SURFACE_WITH_KNOTS((4,2,4),(3,3),(0.,0.000256915317531256,0.000513830635062513),
(0.,1.),.UNSPECIFIED.)
GEOMETRIC_REPRESENTATION_ITEM()
RATIONAL_B_SPLINE_SURFACE(((1.,0.705585838031439,1.),(1.,0.75090243354274,
1.),(1.,0.792329530082544,1.),(1.,0.854288401594183,1.),(1.,0.874998031125163,
1.),(1.,0.874619707139398,1.)))
REPRESENTATION_ITEM('')
SURFACE()
);
#3472=(
BOUNDED_SURFACE()
B_SPLINE_SURFACE(3,2,((#245025,#245026,#245027),(#245028,#245029,#245030),
(#245031,#245032,#245033),(#245034,#245035,#245036),(#245037,#245038,#245039),
(#245040,#245041,#245042)),.UNSPECIFIED.,.F.,.F.,.F.)
B_SPLINE_SURFACE_WITH_KNOTS((4,2,4),(3,3),(0.,0.000256592814262157,0.000513185628524315),
(0.,1.),.UNSPECIFIED.)
GEOMETRIC_REPRESENTATION_ITEM()
RATIONAL_B_SPLINE_SURFACE(((1.,0.708712527163663,1.),(1.,0.75378090261347,
1.),(1.,0.794538995769367,1.),(1.,0.855070770330937,1.),(1.,0.875018427445453,
1.),(1.,0.874619707139386,1.)))
REPRESENTATION_ITEM('')
SURFACE()
);
#3473=(
BOUNDED_SURFACE()
B_SPLINE_SURFACE(3,2,((#245044,#245045,#245046),(#245047,#245048,#245049),
(#245050,#245051,#245052),(#245053,#245054,#245055)),.UNSPECIFIED.,.F.,
 .F.,.F.)
B_SPLINE_SURFACE_WITH_KNOTS((4,4),(3,3),(0.,0.000511815072430399),(0.,1.0010559836589),
 .UNSPECIFIED.)
GEOMETRIC_REPRESENTATION_ITEM()
RATIONAL_B_SPLINE_SURFACE(((1.,0.706797490733676,1.00061923411707),(1.,
0.706182062146617,1.00062053388213),(1.,0.705584062768934,1.00062179683727),
(1.,0.705266224770433,1.00062246810074)))
REPRESENTATION_ITEM('')
SURFACE()
);
#3474=(
BOUNDED_SURFACE()
B_SPLINE_SURFACE(3,2,((#245061,#245062,#245063),(#245064,#245065,#245066),
(#245067,#245068,#245069),(#245070,#245071,#245072),(#245073,#245074,#245075),
(#245076,#245077,#245078)),.UNSPECIFIED.,.F.,.F.,.F.)
B_SPLINE_SURFACE_WITH_KNOTS((4,2,4),(3,3),(-3.1712913545201E-18,0.000257652232350882,
0.000515304464701766),(0.,1.),.UNSPECIFIED.)
GEOMETRIC_REPRESENTATION_ITEM()
RATIONAL_B_SPLINE_SURFACE(((1.,0.874619707139392,1.),(1.,0.874861180430489,
1.),(1.,0.855455725921166,1.),(1.,0.794699358954979,1.),(1.,0.75376897778886,
1.),(1.,0.708712527163655,1.)))
REPRESENTATION_ITEM('')
SURFACE()
);
#3475=(
BOUNDED_SURFACE()
B_SPLINE_SURFACE(3,2,((#245084,#245085,#245086),(#245087,#245088,#245089),
(#245090,#245091,#245092),(#245093,#245094,#245095)),.UNSPECIFIED.,.F.,
 .F.,.F.)
B_SPLINE_SURFACE_WITH_KNOTS((4,4),(3,3),(2.71050543121376E-20,0.000397394373651917),
(0.,1.),.UNSPECIFIED.)
GEOMETRIC_REPRESENTATION_ITEM()
RATIONAL_B_SPLINE_SURFACE(((1.,0.707106781186545,1.),(1.,0.707752587915855,
1.),(1.,0.70837765454072,1.),(1.,0.708689770883334,1.)))
REPRESENTATION_ITEM('')
SURFACE()
);
#3476=(
BOUNDED_SURFACE()
B_SPLINE_SURFACE(3,2,((#245097,#245098,#245099),(#245100,#245101,#245102),
(#245103,#245104,#245105),(#245106,#245107,#245108)),.UNSPECIFIED.,.F.,
 .F.,.F.)
B_SPLINE_SURFACE_WITH_KNOTS((4,4),(3,3),(0.,0.000511815456479795),(0.,1.00105873159796),
 .UNSPECIFIED.)
GEOMETRIC_REPRESENTATION_ITEM()
RATIONAL_B_SPLINE_SURFACE(((1.,0.708394529056934,1.00061746385245),(1.,
0.708058564167418,1.00061817524574),(1.,0.707430835372665,1.00061950443836),
(1.,0.706796685880961,1.00062084722657)))
REPRESENTATION_ITEM('')
SURFACE()
);
#3477=(
BOUNDED_SURFACE()
B_SPLINE_SURFACE(3,2,((#245114,#245115,#245116),(#245117,#245118,#245119),
(#245120,#245121,#245122),(#245123,#245124,#245125)),.UNSPECIFIED.,.F.,
 .F.,.F.)
B_SPLINE_SURFACE_WITH_KNOTS((4,4),(3,3),(0.,0.000397394465448323),(0.,1.),
 .UNSPECIFIED.)
GEOMETRIC_REPRESENTATION_ITEM()
RATIONAL_B_SPLINE_SURFACE(((1.,0.705498956110748,1.),(1.,0.705821764811774,
1.),(1.,0.706461952521149,1.),(1.,0.707106781186538,1.)))
REPRESENTATION_ITEM('')
SURFACE()
);
#3478=(
BOUNDED_SURFACE()
B_SPLINE_SURFACE(3,2,((#245131,#245132,#245133),(#245134,#245135,#245136),
(#245137,#245138,#245139),(#245140,#245141,#245142)),.UNSPECIFIED.,.F.,
 .F.,.F.)
B_SPLINE_SURFACE_WITH_KNOTS((4,4),(3,3),(0.,0.000397394410828735),(0.,1.),
 .UNSPECIFIED.)
GEOMETRIC_REPRESENTATION_ITEM()
RATIONAL_B_SPLINE_SURFACE(((1.,0.708689770883322,1.),(1.,0.708376440034484,
1.),(1.,0.707750498698409,1.),(1.,0.70710678118656,1.)))
REPRESENTATION_ITEM('')
SURFACE()
);
#3479=(
BOUNDED_SURFACE()
B_SPLINE_SURFACE(3,2,((#245148,#245149,#245150),(#245151,#245152,#245153),
(#245154,#245155,#245156),(#245157,#245158,#245159)),.UNSPECIFIED.,.F.,
 .F.,.F.)
B_SPLINE_SURFACE_WITH_KNOTS((4,4),(3,3),(0.,0.000511815090126181),(0.,1.00105592270304),
 .UNSPECIFIED.)
GEOMETRIC_REPRESENTATION_ITEM()
RATIONAL_B_SPLINE_SURFACE(((1.,0.705266242717251,1.00062243213133),(1.,
0.705584085908867,1.00062176089565),(1.,0.706182089450269,1.00062049800462),
(1.,0.706797508587227,1.00061919833454)))
REPRESENTATION_ITEM('')
SURFACE()
);
#3480=(
BOUNDED_SURFACE()
B_SPLINE_SURFACE(3,2,((#245161,#245162,#245163),(#245164,#245165,#245166),
(#245167,#245168,#245169),(#245170,#245171,#245172)),.UNSPECIFIED.,.F.,
 .F.,.F.)
B_SPLINE_SURFACE_WITH_KNOTS((4,4),(3,3),(0.,0.000397394428086618),(0.,1.),
 .UNSPECIFIED.)
GEOMETRIC_REPRESENTATION_ITEM()
RATIONAL_B_SPLINE_SURFACE(((1.,0.707106781186571,1.),(1.,0.706459846759077,
1.),(1.,0.705820510737271,1.),(1.,0.705498956110762,1.)))
REPRESENTATION_ITEM('')
SURFACE()
);
#3481=(
BOUNDED_SURFACE()
B_SPLINE_SURFACE(3,2,((#245178,#245179,#245180),(#245181,#245182,#245183),
(#245184,#245185,#245186),(#245187,#245188,#245189),(#245190,#245191,#245192),
(#245193,#245194,#245195)),.UNSPECIFIED.,.F.,.F.,.F.)
B_SPLINE_SURFACE_WITH_KNOTS((4,2,4),(3,3),(5.01443504774546E-19,0.000257953807872845,
0.00051590761574569),(0.,1.),.UNSPECIFIED.)
GEOMETRIC_REPRESENTATION_ITEM()
RATIONAL_B_SPLINE_SURFACE(((1.,0.874619707139404,1.),(1.,0.874834349678571,
1.),(1.,0.854686104158358,1.),(1.,0.792476597914571,1.),(1.,0.750887854595536,
1.),(1.,0.705585838031444,1.)))
REPRESENTATION_ITEM('')
SURFACE()
);
#3482=(
BOUNDED_SURFACE()
B_SPLINE_SURFACE(3,2,((#245201,#245202,#245203),(#245204,#245205,#245206),
(#245207,#245208,#245209),(#245210,#245211,#245212)),.UNSPECIFIED.,.F.,
 .F.,.F.)
B_SPLINE_SURFACE_WITH_KNOTS((4,4),(3,3),(0.,0.000511815437699152),(0.,1.00105881331367),
 .UNSPECIFIED.)
GEOMETRIC_REPRESENTATION_ITEM()
RATIONAL_B_SPLINE_SURFACE(((1.,0.706796661946975,1.00062089519589),(1.,
0.707430821225895,1.00061955228331),(1.,0.708058545831334,1.00061822299697),
(1.,0.708394505253363,1.00061751156035)))
REPRESENTATION_ITEM('')
SURFACE()
);
#3483=(
BOUNDED_SURFACE()
B_SPLINE_SURFACE(3,2,((#245214,#245215,#245216),(#245217,#245218,#245219),
(#245220,#245221,#245222),(#245223,#245224,#245225),(#245226,#245227,#245228),
(#245229,#245230,#245231)),.UNSPECIFIED.,.F.,.F.,.F.)
B_SPLINE_SURFACE_WITH_KNOTS((4,2,4),(3,3),(-2.84603070277445E-18,0.000256915317531263,
0.000513830635062529),(0.,1.),.UNSPECIFIED.)
GEOMETRIC_REPRESENTATION_ITEM()
RATIONAL_B_SPLINE_SURFACE(((1.,0.705585838031451,1.),(1.,0.750902433542774,
1.),(1.,0.792329530082481,1.),(1.,0.854288401594243,1.),(1.,0.87499803112512,
1.),(1.,0.874619707139395,1.)))
REPRESENTATION_ITEM('')
SURFACE()
);
#3484=(
BOUNDED_SURFACE()
B_SPLINE_SURFACE(3,2,((#245237,#245238,#245239),(#245240,#245241,#245242),
(#245243,#245244,#245245),(#245246,#245247,#245248),(#245249,#245250,#245251),
(#245252,#245253,#245254)),.UNSPECIFIED.,.F.,.F.,.F.)
B_SPLINE_SURFACE_WITH_KNOTS((4,2,4),(3,3),(-1.09233368877915E-17,0.000256592814262153,
0.000513185628524316),(0.,1.),.UNSPECIFIED.)
GEOMETRIC_REPRESENTATION_ITEM()
RATIONAL_B_SPLINE_SURFACE(((1.,0.708712527163668,1.),(1.,0.753780902613415,
1.),(1.,0.794538995769434,1.),(1.,0.855070770330872,1.),(1.,0.875018427445518,
1.),(1.,0.874619707139395,1.)))
REPRESENTATION_ITEM('')
SURFACE()
);
#3485=(
BOUNDED_SURFACE()
B_SPLINE_SURFACE(3,2,((#245256,#245257,#245258),(#245259,#245260,#245261),
(#245262,#245263,#245264),(#245265,#245266,#245267)),.UNSPECIFIED.,.F.,
 .F.,.F.)
B_SPLINE_SURFACE_WITH_KNOTS((4,4),(3,3),(0.,0.000511815072430409),(0.,1.0010559836586),
 .UNSPECIFIED.)
GEOMETRIC_REPRESENTATION_ITEM()
RATIONAL_B_SPLINE_SURFACE(((1.,0.706797490733765,1.00061923411689),(1.,
0.706182062146697,1.00062053388195),(1.,0.705584062769033,1.00062179683709),
(1.,0.705266224770523,1.00062246810056)))
REPRESENTATION_ITEM('')
SURFACE()
);
#3486=(
BOUNDED_SURFACE()
B_SPLINE_SURFACE(3,2,((#245273,#245274,#245275),(#245276,#245277,#245278),
(#245279,#245280,#245281),(#245282,#245283,#245284),(#245285,#245286,#245287),
(#245288,#245289,#245290)),.UNSPECIFIED.,.F.,.F.,.F.)
B_SPLINE_SURFACE_WITH_KNOTS((4,2,4),(3,3),(-9.52742659071637E-18,0.000257652232350881,
0.000515304464701771),(0.,1.),.UNSPECIFIED.)
GEOMETRIC_REPRESENTATION_ITEM()
RATIONAL_B_SPLINE_SURFACE(((1.,0.874619707139396,1.),(1.,0.874861180430588,
1.),(1.,0.855455725921017,1.),(1.,0.794699358955082,1.),(1.,0.753768977788791,
1.),(1.,0.70871252716365,1.)))
REPRESENTATION_ITEM('')
SURFACE()
);
#3487=(
BOUNDED_SURFACE()
B_SPLINE_SURFACE(3,2,((#245296,#245297,#245298),(#245299,#245300,#245301),
(#245302,#245303,#245304),(#245305,#245306,#245307)),.UNSPECIFIED.,.F.,
 .F.,.F.)
B_SPLINE_SURFACE_WITH_KNOTS((4,4),(3,3),(-5.96311194867027E-19,0.000397394373651909),
(0.,1.),.UNSPECIFIED.)
GEOMETRIC_REPRESENTATION_ITEM()
RATIONAL_B_SPLINE_SURFACE(((1.,0.707106781186546,1.),(1.,0.707752587915895,
1.),(1.,0.708377654540719,1.),(1.,0.70868977088333,1.)))
REPRESENTATION_ITEM('')
SURFACE()
);
#3488=(
BOUNDED_SURFACE()
B_SPLINE_SURFACE(3,2,((#245309,#245310,#245311),(#245312,#245313,#245314),
(#245315,#245316,#245317),(#245318,#245319,#245320)),.UNSPECIFIED.,.F.,
 .F.,.F.)
B_SPLINE_SURFACE_WITH_KNOTS((4,4),(3,3),(0.,0.000511815456479797),(0.,1.00105873159678),
 .UNSPECIFIED.)
GEOMETRIC_REPRESENTATION_ITEM()
RATIONAL_B_SPLINE_SURFACE(((1.,0.708394529057283,1.00061746385176),(1.,
0.70805856416776,1.00061817524505),(1.,0.707430835373029,1.00061950443767),
(1.,0.706796685881307,1.00062084722587)))
REPRESENTATION_ITEM('')
SURFACE()
);
#3489=(
BOUNDED_SURFACE()
B_SPLINE_SURFACE(3,2,((#245326,#245327,#245328),(#245329,#245330,#245331),
(#245332,#245333,#245334),(#245335,#245336,#245337)),.UNSPECIFIED.,.F.,
 .F.,.F.)
B_SPLINE_SURFACE_WITH_KNOTS((4,4),(3,3),(0.,0.00039739446544831),(0.,1.),
 .UNSPECIFIED.)
GEOMETRIC_REPRESENTATION_ITEM()
RATIONAL_B_SPLINE_SURFACE(((1.,0.705498956110735,1.),(1.,0.705821764811779,
1.),(1.,0.70646195252112,1.),(1.,0.707106781186562,1.)))
REPRESENTATION_ITEM('')
SURFACE()
);
#3490=(
BOUNDED_SURFACE()
B_SPLINE_SURFACE(3,2,((#245343,#245344,#245345),(#245346,#245347,#245348),
(#245349,#245350,#245351),(#245352,#245353,#245354)),.UNSPECIFIED.,.F.,
 .F.,.F.)
B_SPLINE_SURFACE_WITH_KNOTS((4,4),(3,3),(0.,0.000397394410828739),(0.,1.),
 .UNSPECIFIED.)
GEOMETRIC_REPRESENTATION_ITEM()
RATIONAL_B_SPLINE_SURFACE(((1.,0.708689770883341,1.),(1.,0.708376440034489,
1.),(1.,0.70775049869842,1.),(1.,0.707106781186549,1.)))
REPRESENTATION_ITEM('')
SURFACE()
);
#3491=(
BOUNDED_SURFACE()
B_SPLINE_SURFACE(3,2,((#245360,#245361,#245362),(#245363,#245364,#245365),
(#245366,#245367,#245368),(#245369,#245370,#245371)),.UNSPECIFIED.,.F.,
 .F.,.F.)
B_SPLINE_SURFACE_WITH_KNOTS((4,4),(3,3),(-1.59919820441612E-18,0.000511815090126168),
(0.,1.00105592270431),.UNSPECIFIED.)
GEOMETRIC_REPRESENTATION_ITEM()
RATIONAL_B_SPLINE_SURFACE(((1.,0.705266242716864,1.00062243213208),(1.,
0.705584085908508,1.0006217608964),(1.,0.706182089449863,1.00062049800537),
(1.,0.706797508586865,1.00061919833529)))
REPRESENTATION_ITEM('')
SURFACE()
);
#3492=(
BOUNDED_SURFACE()
B_SPLINE_SURFACE(3,2,((#245373,#245374,#245375),(#245376,#245377,#245378),
(#245379,#245380,#245381),(#245382,#245383,#245384)),.UNSPECIFIED.,.F.,
 .F.,.F.)
B_SPLINE_SURFACE_WITH_KNOTS((4,4),(3,3),(0.,0.00039739442808662),(0.,1.),
 .UNSPECIFIED.)
GEOMETRIC_REPRESENTATION_ITEM()
RATIONAL_B_SPLINE_SURFACE(((1.,0.707106781186562,1.),(1.,0.706459846759107,
1.),(1.,0.705820510737251,1.),(1.,0.705498956110768,1.)))
REPRESENTATION_ITEM('')
SURFACE()
);
#3493=(
BOUNDED_SURFACE()
B_SPLINE_SURFACE(3,2,((#245390,#245391,#245392),(#245393,#245394,#245395),
(#245396,#245397,#245398),(#245399,#245400,#245401),(#245402,#245403,#245404),
(#245405,#245406,#245407)),.UNSPECIFIED.,.F.,.F.,.F.)
B_SPLINE_SURFACE_WITH_KNOTS((4,2,4),(3,3),(0.,0.000257953807872846,0.000515907615745693),
(0.,1.),.UNSPECIFIED.)
GEOMETRIC_REPRESENTATION_ITEM()
RATIONAL_B_SPLINE_SURFACE(((1.,0.874619707139391,1.),(1.,0.874834349679018,
1.),(1.,0.854686104157766,1.),(1.,0.792476597915161,1.),(1.,0.75088785459512,
1.),(1.,0.705585838031422,1.)))
REPRESENTATION_ITEM('')
SURFACE()
);
#3494=(
BOUNDED_SURFACE()
B_SPLINE_SURFACE(3,2,((#245413,#245414,#245415),(#245416,#245417,#245418),
(#245419,#245420,#245421),(#245422,#245423,#245424)),.UNSPECIFIED.,.F.,
 .F.,.F.)
B_SPLINE_SURFACE_WITH_KNOTS((4,4),(3,3),(-5.42101086242752E-20,0.000511815437699146),
(0.,1.00105881331879),.UNSPECIFIED.)
GEOMETRIC_REPRESENTATION_ITEM()
RATIONAL_B_SPLINE_SURFACE(((1.,0.706796661945487,1.00062089519889),(1.,
0.707430821224365,1.00061955228631),(1.,0.708058545829886,1.00061822299996),
(1.,0.708394505251882,1.00061751156334)))
REPRESENTATION_ITEM('')
SURFACE()
);
#3495=(
BOUNDED_SURFACE()
B_SPLINE_SURFACE(3,2,((#245426,#245427,#245428),(#245429,#245430,#245431),
(#245432,#245433,#245434),(#245435,#245436,#245437),(#245438,#245439,#245440),
(#245441,#245442,#245443)),.UNSPECIFIED.,.F.,.F.,.F.)
B_SPLINE_SURFACE_WITH_KNOTS((4,2,4),(3,3),(0.,0.000256915317531259,0.000513830635062518),
(0.,1.),.UNSPECIFIED.)
GEOMETRIC_REPRESENTATION_ITEM()
RATIONAL_B_SPLINE_SURFACE(((1.,0.705585838031442,1.),(1.,0.750902433542966,
1.),(1.,0.792329530082241,1.),(1.,0.854288401594463,1.),(1.,0.874998031124932,
1.),(1.,0.874619707139397,1.)))
REPRESENTATION_ITEM('')
SURFACE()
);
#3496=(
BOUNDED_SURFACE()
B_SPLINE_SURFACE(3,2,((#245449,#245450,#245451),(#245452,#245453,#245454),
(#245455,#245456,#245457),(#245458,#245459,#245460),(#245461,#245462,#245463),
(#245464,#245465,#245466)),.UNSPECIFIED.,.F.,.F.,.F.)
B_SPLINE_SURFACE_WITH_KNOTS((4,2,4),(3,3),(-1.05709711817337E-18,0.000256592814262156,
0.000513185628524313),(0.,1.),.UNSPECIFIED.)
GEOMETRIC_REPRESENTATION_ITEM()
RATIONAL_B_SPLINE_SURFACE(((1.,0.708712527163677,1.),(1.,0.753780902613637,
1.),(1.,0.79453899576914,1.),(1.,0.855070770331177,1.),(1.,0.875018427445286,
1.),(1.,0.874619707139395,1.)))
REPRESENTATION_ITEM('')
SURFACE()
);
#3497=(
BOUNDED_SURFACE()
B_SPLINE_SURFACE(3,2,((#245468,#245469,#245470),(#245471,#245472,#245473),
(#245474,#245475,#245476),(#245477,#245478,#245479)),.UNSPECIFIED.,.F.,
 .F.,.F.)
B_SPLINE_SURFACE_WITH_KNOTS((4,4),(3,3),(-1.35525271560688E-19,0.000511815072430405),
(0.,1.00105598365711),.UNSPECIFIED.)
GEOMETRIC_REPRESENTATION_ITEM()
RATIONAL_B_SPLINE_SURFACE(((1.,0.706797490734201,1.00061923411602),(1.,
0.706182062147124,1.00062053388108),(1.,0.705584062769492,1.00062179683622),
(1.,0.705266224770974,1.00062246809968)))
REPRESENTATION_ITEM('')
SURFACE()
);
#3498=(
BOUNDED_SURFACE()
B_SPLINE_SURFACE(3,2,((#245485,#245486,#245487),(#245488,#245489,#245490),
(#245491,#245492,#245493),(#245494,#245495,#245496),(#245497,#245498,#245499),
(#245500,#245501,#245502)),.UNSPECIFIED.,.F.,.F.,.F.)
B_SPLINE_SURFACE_WITH_KNOTS((4,2,4),(3,3),(0.,0.000257652232350885,0.00051530446470177),
(0.,1.),.UNSPECIFIED.)
GEOMETRIC_REPRESENTATION_ITEM()
RATIONAL_B_SPLINE_SURFACE(((1.,0.874619707139392,1.),(1.,0.874861180429708,
1.),(1.,0.855455725922225,1.),(1.,0.794699358953907,1.),(1.,0.753768977789676,
1.),(1.,0.70871252716366,1.)))
REPRESENTATION_ITEM('')
SURFACE()
);
#3499=(
BOUNDED_SURFACE()
B_SPLINE_SURFACE(3,2,((#245508,#245509,#245510),(#245511,#245512,#245513),
(#245514,#245515,#245516),(#245517,#245518,#245519)),.UNSPECIFIED.,.F.,
 .F.,.F.)
B_SPLINE_SURFACE_WITH_KNOTS((4,4),(3,3),(-1.5748036555352E-17,0.000397394373651906),
(0.,1.),.UNSPECIFIED.)
GEOMETRIC_REPRESENTATION_ITEM()
RATIONAL_B_SPLINE_SURFACE(((1.,0.707106781186546,1.),(1.,0.70775258791588,
1.),(1.,0.708377654540694,1.),(1.,0.708689770883323,1.)))
REPRESENTATION_ITEM('')
SURFACE()
);
#3500=(
BOUNDED_SURFACE()
B_SPLINE_SURFACE(3,2,((#245521,#245522,#245523),(#245524,#245525,#245526),
(#245527,#245528,#245529),(#245530,#245531,#245532)),.UNSPECIFIED.,.F.,
 .F.,.F.)
B_SPLINE_SURFACE_WITH_KNOTS((4,4),(3,3),(0.,0.000511815456479801),(0.,1.00105873159925),
 .UNSPECIFIED.)
GEOMETRIC_REPRESENTATION_ITEM()
RATIONAL_B_SPLINE_SURFACE(((1.,0.708394529056526,1.00061746385321),(1.,
0.708058564167044,1.0006181752465),(1.,0.707430835372304,1.00061950443912),
(1.,0.706796685880582,1.00062084722733)))
REPRESENTATION_ITEM('')
SURFACE()
);
#3501=(
BOUNDED_SURFACE()
B_SPLINE_SURFACE(3,2,((#245538,#245539,#245540),(#245541,#245542,#245543),
(#245544,#245545,#245546),(#245547,#245548,#245549)),.UNSPECIFIED.,.F.,
 .F.,.F.)
B_SPLINE_SURFACE_WITH_KNOTS((4,4),(3,3),(0.,0.000397394465448322),(0.,1.),
 .UNSPECIFIED.)
GEOMETRIC_REPRESENTATION_ITEM()
RATIONAL_B_SPLINE_SURFACE(((1.,0.705498956110752,1.),(1.,0.705821764811804,
1.),(1.,0.70646195252111,1.),(1.,0.707106781186559,1.)))
REPRESENTATION_ITEM('')
SURFACE()
);
#3502=(
BOUNDED_SURFACE()
B_SPLINE_SURFACE(3,2,((#245555,#245556,#245557),(#245558,#245559,#245560),
(#245561,#245562,#245563),(#245564,#245565,#245566)),.UNSPECIFIED.,.F.,
 .F.,.F.)
B_SPLINE_SURFACE_WITH_KNOTS((4,4),(3,3),(0.,0.00039739441082872),(0.,1.),
 .UNSPECIFIED.)
GEOMETRIC_REPRESENTATION_ITEM()
RATIONAL_B_SPLINE_SURFACE(((1.,0.708689770883314,1.),(1.,0.708376440034513,
1.),(1.,0.70775049869841,1.),(1.,0.707106781186537,1.)))
REPRESENTATION_ITEM('')
SURFACE()
);
#3503=(
BOUNDED_SURFACE()
B_SPLINE_SURFACE(3,2,((#245572,#245573,#245574),(#245575,#245576,#245577),
(#245578,#245579,#245580),(#245581,#245582,#245583)),.UNSPECIFIED.,.F.,
 .F.,.F.)
B_SPLINE_SURFACE_WITH_KNOTS((4,4),(3,3),(0.,0.000511815090126186),(0.,1.00105592270166),
 .UNSPECIFIED.)
GEOMETRIC_REPRESENTATION_ITEM()
RATIONAL_B_SPLINE_SURFACE(((1.,0.705266242717654,1.00062243213052),(1.,
0.705584085909304,1.00062176089484),(1.,0.706182089450655,1.00062049800381),
(1.,0.706797508587642,1.00061919833373)))
REPRESENTATION_ITEM('')
SURFACE()
);
#3504=(
BOUNDED_SURFACE()
B_SPLINE_SURFACE(3,2,((#245585,#245586,#245587),(#245588,#245589,#245590),
(#245591,#245592,#245593),(#245594,#245595,#245596)),.UNSPECIFIED.,.F.,
 .F.,.F.)
B_SPLINE_SURFACE_WITH_KNOTS((4,4),(3,3),(-1.458251921993E-17,0.000397394428086608),
(0.,1.),.UNSPECIFIED.)
GEOMETRIC_REPRESENTATION_ITEM()
RATIONAL_B_SPLINE_SURFACE(((1.,0.707106781186551,1.),(1.,0.70645984675909,
1.),(1.,0.705820510737285,1.),(1.,0.705498956110753,1.)))
REPRESENTATION_ITEM('')
SURFACE()
);
#3505=(
BOUNDED_SURFACE()
B_SPLINE_SURFACE(3,2,((#245602,#245603,#245604),(#245605,#245606,#245607),
(#245608,#245609,#245610),(#245611,#245612,#245613),(#245614,#245615,#245616),
(#245617,#245618,#245619)),.UNSPECIFIED.,.F.,.F.,.F.)
B_SPLINE_SURFACE_WITH_KNOTS((4,2,4),(3,3),(0.,0.00025795380787285,0.000515907615745699),
(0.,1.),.UNSPECIFIED.)
GEOMETRIC_REPRESENTATION_ITEM()
RATIONAL_B_SPLINE_SURFACE(((1.,0.874619707139398,1.),(1.,0.874834349678536,
1.),(1.,0.854686104158402,1.),(1.,0.792476597914546,1.),(1.,0.7508878545956,
1.),(1.,0.705585838031444,1.)))
REPRESENTATION_ITEM('')
SURFACE()
);
#3506=(
BOUNDED_SURFACE()
B_SPLINE_SURFACE(3,2,((#245625,#245626,#245627),(#245628,#245629,#245630),
(#245631,#245632,#245633),(#245634,#245635,#245636)),.UNSPECIFIED.,.F.,
 .F.,.F.)
B_SPLINE_SURFACE_WITH_KNOTS((4,4),(3,3),(-5.6920614055489E-19,0.000511815437699162),
(0.,1.00105881331531),.UNSPECIFIED.)
GEOMETRIC_REPRESENTATION_ITEM()
RATIONAL_B_SPLINE_SURFACE(((1.,0.706796661946493,1.00062089519685),(1.,
0.707430821225386,1.00061955228427),(1.,0.708058545830895,1.00061822299793),
(1.,0.70839450525288,1.00061751156131)))
REPRESENTATION_ITEM('')
SURFACE()
);
#3507=(
BOUNDED_SURFACE()
B_SPLINE_SURFACE(3,2,((#245638,#245639,#245640),(#245641,#245642,#245643),
(#245644,#245645,#245646),(#245647,#245648,#245649),(#245650,#245651,#245652),
(#245653,#245654,#245655)),.UNSPECIFIED.,.F.,.F.,.F.)
B_SPLINE_SURFACE_WITH_KNOTS((4,2,4),(3,3),(0.,0.000256915317531261,0.000513830635062522),
(0.,1.),.UNSPECIFIED.)
GEOMETRIC_REPRESENTATION_ITEM()
RATIONAL_B_SPLINE_SURFACE(((1.,0.705585838031423,1.),(1.,0.750902433542322,
1.),(1.,0.792329530083111,1.),(1.,0.854288401593614,1.),(1.,0.874998031125594,
1.),(1.,0.874619707139391,1.)))
REPRESENTATION_ITEM('')
SURFACE()
);
#3508=(
BOUNDED_SURFACE()
B_SPLINE_SURFACE(3,2,((#245661,#245662,#245663),(#245664,#245665,#245666),
(#245667,#245668,#245669),(#245670,#245671,#245672),(#245673,#245674,#245675),
(#245676,#245677,#245678)),.UNSPECIFIED.,.F.,.F.,.F.)
B_SPLINE_SURFACE_WITH_KNOTS((4,2,4),(3,3),(-9.86623976961809E-18,0.000256592814262149,
0.000513185628524309),(0.,1.),.UNSPECIFIED.)
GEOMETRIC_REPRESENTATION_ITEM()
RATIONAL_B_SPLINE_SURFACE(((1.,0.708712527163638,1.),(1.,0.753780902613253,
1.),(1.,0.794538995769658,1.),(1.,0.855070770330655,1.),(1.,0.875018427445672,
1.),(1.,0.874619707139396,1.)))
REPRESENTATION_ITEM('')
SURFACE()
);
#3509=(
BOUNDED_SURFACE()
B_SPLINE_SURFACE(3,2,((#245680,#245681,#245682),(#245683,#245684,#245685),
(#245686,#245687,#245688),(#245689,#245690,#245691)),.UNSPECIFIED.,.F.,
 .F.,.F.)
B_SPLINE_SURFACE_WITH_KNOTS((4,4),(3,3),(5.42101086242752E-19,0.000511815072430404),
(0.,1.00105598366058),.UNSPECIFIED.)
GEOMETRIC_REPRESENTATION_ITEM()
RATIONAL_B_SPLINE_SURFACE(((1.,0.706797490733183,1.00061923411805),(1.,
0.706182062146105,1.00062053388312),(1.,0.705584062768457,1.00062179683826),
(1.,0.705266224769939,1.00062246810173)))
REPRESENTATION_ITEM('')
SURFACE()
);
#3510=(
BOUNDED_SURFACE()
B_SPLINE_SURFACE(3,2,((#245697,#245698,#245699),(#245700,#245701,#245702),
(#245703,#245704,#245705),(#245706,#245707,#245708),(#245709,#245710,#245711),
(#245712,#245713,#245714)),.UNSPECIFIED.,.F.,.F.,.F.)
B_SPLINE_SURFACE_WITH_KNOTS((4,2,4),(3,3),(-5.16351284646221E-18,0.000257652232350889,
0.000515304464701783),(0.,1.),.UNSPECIFIED.)
GEOMETRIC_REPRESENTATION_ITEM()
RATIONAL_B_SPLINE_SURFACE(((1.,0.874619707139395,1.),(1.,0.874861180431115,
1.),(1.,0.855455725920305,1.),(1.,0.794699358955837,1.),(1.,0.753768977788197,
1.),(1.,0.708712527163675,1.)))
REPRESENTATION_ITEM('')
SURFACE()
);
#3511=(
BOUNDED_SURFACE()
B_SPLINE_SURFACE(3,2,((#245720,#245721,#245722),(#245723,#245724,#245725),
(#245726,#245727,#245728),(#245729,#245730,#245731)),.UNSPECIFIED.,.F.,
 .F.,.F.)
B_SPLINE_SURFACE_WITH_KNOTS((4,4),(3,3),(0.,0.000397394373651917),(0.,1.),
 .UNSPECIFIED.)
GEOMETRIC_REPRESENTATION_ITEM()
RATIONAL_B_SPLINE_SURFACE(((1.,0.707106781186532,1.),(1.,0.707752587915907,
1.),(1.,0.708377654540682,1.),(1.,0.708689770883325,1.)))
REPRESENTATION_ITEM('')
SURFACE()
);
#3512=(
BOUNDED_SURFACE()
B_SPLINE_SURFACE(3,2,((#245733,#245734,#245735),(#245736,#245737,#245738),
(#245739,#245740,#245741),(#245742,#245743,#245744)),.UNSPECIFIED.,.F.,
 .F.,.F.)
B_SPLINE_SURFACE_WITH_KNOTS((4,4),(3,3),(-2.41234983378025E-18,0.000511815456479792),
(0.,1.00105873159715),.UNSPECIFIED.)
GEOMETRIC_REPRESENTATION_ITEM()
RATIONAL_B_SPLINE_SURFACE(((1.,0.708394529057139,1.00061746385198),(1.,
0.708058564167716,1.00061817524526),(1.,0.707430835372875,1.00061950443788),
(1.,0.706796685881197,1.00062084722609)))
REPRESENTATION_ITEM('')
SURFACE()
);
#3513=(
BOUNDED_SURFACE()
B_SPLINE_SURFACE(3,2,((#245750,#245751,#245752),(#245753,#245754,#245755),
(#245756,#245757,#245758),(#245759,#245760,#245761)),.UNSPECIFIED.,.F.,
 .F.,.F.)
B_SPLINE_SURFACE_WITH_KNOTS((4,4),(3,3),(-2.84603070277445E-18,0.000397394465448296),
(0.,1.),.UNSPECIFIED.)
GEOMETRIC_REPRESENTATION_ITEM()
RATIONAL_B_SPLINE_SURFACE(((1.,0.705498956110741,1.),(1.,0.70582176481181,
1.),(1.,0.706461952521106,1.),(1.,0.707106781186558,1.)))
REPRESENTATION_ITEM('')
SURFACE()
);
#3514=(
BOUNDED_SURFACE()
B_SPLINE_SURFACE(3,2,((#245767,#245768,#245769),(#245770,#245771,#245772),
(#245773,#245774,#245775),(#245776,#245777,#245778)),.UNSPECIFIED.,.F.,
 .F.,.F.)
B_SPLINE_SURFACE_WITH_KNOTS((4,4),(3,3),(0.,0.000397394410828738),(0.,1.),
 .UNSPECIFIED.)
GEOMETRIC_REPRESENTATION_ITEM()
RATIONAL_B_SPLINE_SURFACE(((1.,0.708689770883334,1.),(1.,0.708376440034488,
1.),(1.,0.707750498698412,1.),(1.,0.70710678118655,1.)))
REPRESENTATION_ITEM('')
SURFACE()
);
#3515=(
BOUNDED_SURFACE()
B_SPLINE_SURFACE(3,2,((#245784,#245785,#245786),(#245787,#245788,#245789),
(#245790,#245791,#245792),(#245793,#245794,#245795)),.UNSPECIFIED.,.F.,
 .F.,.F.)
B_SPLINE_SURFACE_WITH_KNOTS((4,4),(3,3),(0.,0.000511815090126173),(0.,1.00105592270469),
 .UNSPECIFIED.)
GEOMETRIC_REPRESENTATION_ITEM()
RATIONAL_B_SPLINE_SURFACE(((1.,0.70526624271676,1.00062243213231),(1.,0.705584085908403,
1.00062176089662),(1.,0.706182089449747,1.00062049800559),(1.,0.706797508586756,
1.00061919833551)))
REPRESENTATION_ITEM('')
SURFACE()
);
#3516=(
BOUNDED_SURFACE()
B_SPLINE_SURFACE(3,2,((#245797,#245798,#245799),(#245800,#245801,#245802),
(#245803,#245804,#245805),(#245806,#245807,#245808)),.UNSPECIFIED.,.F.,
 .F.,.F.)
B_SPLINE_SURFACE_WITH_KNOTS((4,4),(3,3),(5.96311194867027E-19,0.000397394428086636),
(0.,1.),.UNSPECIFIED.)
GEOMETRIC_REPRESENTATION_ITEM()
RATIONAL_B_SPLINE_SURFACE(((1.,0.70710678118655,1.),(1.,0.706459846759095,
1.),(1.,0.705820510737291,1.),(1.,0.705498956110747,1.)))
REPRESENTATION_ITEM('')
SURFACE()
);
#3517=(
BOUNDED_SURFACE()
B_SPLINE_SURFACE(3,2,((#245814,#245815,#245816),(#245817,#245818,#245819),
(#245820,#245821,#245822),(#245823,#245824,#245825),(#245826,#245827,#245828),
(#245829,#245830,#245831)),.UNSPECIFIED.,.F.,.F.,.F.)
B_SPLINE_SURFACE_WITH_KNOTS((4,2,4),(3,3),(5.14996031930615E-19,0.000257953807872846,
0.000515907615745692),(0.,1.),.UNSPECIFIED.)
GEOMETRIC_REPRESENTATION_ITEM()
RATIONAL_B_SPLINE_SURFACE(((1.,0.874619707139401,1.),(1.,0.874834349679141,
1.),(1.,0.854686104157596,1.),(1.,0.792476597915346,1.),(1.,0.750887854594966,
1.),(1.,0.705585838031443,1.)))
REPRESENTATION_ITEM('')
SURFACE()
);
#3518=(
BOUNDED_SURFACE()
B_SPLINE_SURFACE(3,2,((#245837,#245838,#245839),(#245840,#245841,#245842),
(#245843,#245844,#245845),(#245846,#245847,#245848)),.UNSPECIFIED.,.F.,
 .F.,.F.)
B_SPLINE_SURFACE_WITH_KNOTS((4,4),(3,3),(0.,0.000511815437699156),(0.,1.00105881331562),
 .UNSPECIFIED.)
GEOMETRIC_REPRESENTATION_ITEM()
RATIONAL_B_SPLINE_SURFACE(((1.,0.706796661946404,1.00062089519703),(1.,
0.707430821225336,1.00061955228445),(1.,0.70805854583075,1.00061822299811),
(1.,0.708394505252815,1.00061751156149)))
REPRESENTATION_ITEM('')
SURFACE()
);
#3519=(
BOUNDED_SURFACE()
B_SPLINE_SURFACE(3,2,((#245850,#245851,#245852),(#245853,#245854,#245855),
(#245856,#245857,#245858),(#245859,#245860,#245861),(#245862,#245863,#245864),
(#245865,#245866,#245867)),.UNSPECIFIED.,.F.,.F.,.F.)
B_SPLINE_SURFACE_WITH_KNOTS((4,2,4),(3,3),(-2.71050543121376E-20,0.000256915317531265,
0.00051383063506253),(0.,1.),.UNSPECIFIED.)
GEOMETRIC_REPRESENTATION_ITEM()
RATIONAL_B_SPLINE_SURFACE(((1.,0.705585838031445,1.),(1.,0.750902433542657,
1.),(1.,0.792329530082642,1.),(1.,0.854288401594088,1.),(1.,0.87499803112522,
1.),(1.,0.874619707139401,1.)))
REPRESENTATION_ITEM('')
SURFACE()
);
#3520=(
BOUNDED_SURFACE()
B_SPLINE_SURFACE(3,2,((#245873,#245874,#245875),(#245876,#245877,#245878),
(#245879,#245880,#245881),(#245882,#245883,#245884),(#245885,#245886,#245887),
(#245888,#245889,#245890)),.UNSPECIFIED.,.F.,.F.,.F.)
B_SPLINE_SURFACE_WITH_KNOTS((4,2,4),(3,3),(1.43656787854329E-18,0.000256592814262158,
0.000513185628524315),(0.,1.),.UNSPECIFIED.)
GEOMETRIC_REPRESENTATION_ITEM()
RATIONAL_B_SPLINE_SURFACE(((1.,0.70871252716365,1.),(1.,0.753780902613447,
1.),(1.,0.794538995769409,1.),(1.,0.855070770330912,1.),(1.,0.875018427445475,
1.),(1.,0.874619707139396,1.)))
REPRESENTATION_ITEM('')
SURFACE()
);
#3521=(
BOUNDED_SURFACE()
B_SPLINE_SURFACE(3,2,((#245892,#245893,#245894),(#245895,#245896,#245897),
(#245898,#245899,#245900),(#245901,#245902,#245903)),.UNSPECIFIED.,.F.,
 .F.,.F.)
B_SPLINE_SURFACE_WITH_KNOTS((4,4),(3,3),(5.96311194867027E-19,0.000511815072430399),
(0.,1.00105598365885),.UNSPECIFIED.)
GEOMETRIC_REPRESENTATION_ITEM()
RATIONAL_B_SPLINE_SURFACE(((1.,0.706797490733679,1.00061923411704),(1.,
0.706182062146613,1.0006205338821),(1.,0.705584062769007,1.00062179683724),
(1.,0.705266224770429,1.00062246810071)))
REPRESENTATION_ITEM('')
SURFACE()
);
#3522=(
BOUNDED_SURFACE()
B_SPLINE_SURFACE(3,2,((#245909,#245910,#245911),(#245912,#245913,#245914),
(#245915,#245916,#245917),(#245918,#245919,#245920),(#245921,#245922,#245923),
(#245924,#245925,#245926)),.UNSPECIFIED.,.F.,.F.,.F.)
B_SPLINE_SURFACE_WITH_KNOTS((4,2,4),(3,3),(0.,0.00025765223235089,0.00051530446470178),
(0.,1.),.UNSPECIFIED.)
GEOMETRIC_REPRESENTATION_ITEM()
RATIONAL_B_SPLINE_SURFACE(((1.,0.874619707139387,1.),(1.,0.874861180430702,
1.),(1.,0.855455725920869,1.),(1.,0.794699358955257,1.),(1.,0.753768977788647,
1.),(1.,0.708712527163647,1.)))
REPRESENTATION_ITEM('')
SURFACE()
);
#3523=(
BOUNDED_SURFACE()
B_SPLINE_SURFACE(3,2,((#245932,#245933,#245934),(#245935,#245936,#245937),
(#245938,#245939,#245940),(#245941,#245942,#245943)),.UNSPECIFIED.,.F.,
 .F.,.F.)
B_SPLINE_SURFACE_WITH_KNOTS((4,4),(3,3),(0.,0.000397394373651909),(0.,1.),
 .UNSPECIFIED.)
GEOMETRIC_REPRESENTATION_ITEM()
RATIONAL_B_SPLINE_SURFACE(((1.,0.707106781186545,1.),(1.,0.707752587915893,
1.),(1.,0.70837765454068,1.),(1.,0.70868977088333,1.)))
REPRESENTATION_ITEM('')
SURFACE()
);
#3524=(
BOUNDED_SURFACE()
B_SPLINE_SURFACE(3,2,((#245945,#245946,#245947),(#245948,#245949,#245950),
(#245951,#245952,#245953),(#245954,#245955,#245956)),.UNSPECIFIED.,.F.,
 .F.,.F.)
B_SPLINE_SURFACE_WITH_KNOTS((4,4),(3,3),(-5.61074624261249E-18,0.000511815456479791),
(0.,1.00105873159595),.UNSPECIFIED.)
GEOMETRIC_REPRESENTATION_ITEM()
RATIONAL_B_SPLINE_SURFACE(((1.,0.708394529057486,1.00061746385128),(1.,
0.708058564168047,1.00061817524457),(1.,0.707430835373218,1.00061950443718),
(1.,0.706796685881535,1.00062084722539)))
REPRESENTATION_ITEM('')
SURFACE()
);
#3525=(
BOUNDED_SURFACE()
B_SPLINE_SURFACE(3,2,((#245962,#245963,#245964),(#245965,#245966,#245967),
(#245968,#245969,#245970),(#245971,#245972,#245973)),.UNSPECIFIED.,.F.,
 .F.,.F.)
B_SPLINE_SURFACE_WITH_KNOTS((4,4),(3,3),(0.,0.000397394465448306),(0.,1.),
 .UNSPECIFIED.)
GEOMETRIC_REPRESENTATION_ITEM()
RATIONAL_B_SPLINE_SURFACE(((1.,0.70549895611075,1.),(1.,0.705821764811804,
1.),(1.,0.706461952521105,1.),(1.,0.707106781186556,1.)))
REPRESENTATION_ITEM('')
SURFACE()
);
#3526=(
BOUNDED_SURFACE()
B_SPLINE_SURFACE(3,2,((#245979,#245980,#245981),(#245982,#245983,#245984),
(#245985,#245986,#245987),(#245988,#245989,#245990)),.UNSPECIFIED.,.F.,
 .F.,.F.)
B_SPLINE_SURFACE_WITH_KNOTS((4,4),(3,3),(-6.23416249179165E-19,0.000397394410828727),
(0.,1.),.UNSPECIFIED.)
GEOMETRIC_REPRESENTATION_ITEM()
RATIONAL_B_SPLINE_SURFACE(((1.,0.70868977088335,1.),(1.,0.708376440034487,
1.),(1.,0.707750498698414,1.),(1.,0.707106781186542,1.)))
REPRESENTATION_ITEM('')
SURFACE()
);
#3527=(
BOUNDED_SURFACE()
B_SPLINE_SURFACE(3,2,((#245996,#245997,#245998),(#245999,#246000,#246001),
(#246002,#246003,#246004),(#246005,#246006,#246007)),.UNSPECIFIED.,.F.,
 .F.,.F.)
B_SPLINE_SURFACE_WITH_KNOTS((4,4),(3,3),(0.,0.000511815090126179),(0.,1.00105592270077),
 .UNSPECIFIED.)
GEOMETRIC_REPRESENTATION_ITEM()
RATIONAL_B_SPLINE_SURFACE(((1.,0.705266242717907,1.00062243212999),(1.,
0.705584085909567,1.00062176089431),(1.,0.706182089450896,1.00062049800328),
(1.,0.706797508587904,1.00061919833321)))
REPRESENTATION_ITEM('')
SURFACE()
);
#3528=(
BOUNDED_SURFACE()
B_SPLINE_SURFACE(3,2,((#246009,#246010,#246011),(#246012,#246013,#246014),
(#246015,#246016,#246017),(#246018,#246019,#246020)),.UNSPECIFIED.,.F.,
 .F.,.F.)
B_SPLINE_SURFACE_WITH_KNOTS((4,4),(3,3),(0.,0.000397394428086625),(0.,1.),
 .UNSPECIFIED.)
GEOMETRIC_REPRESENTATION_ITEM()
RATIONAL_B_SPLINE_SURFACE(((1.,0.70710678118656,1.),(1.,0.706459846759085,
1.),(1.,0.705820510737268,1.),(1.,0.70549895611075,1.)))
REPRESENTATION_ITEM('')
SURFACE()
);
#3529=(
BOUNDED_SURFACE()
B_SPLINE_SURFACE(3,2,((#246026,#246027,#246028),(#246029,#246030,#246031),
(#246032,#246033,#246034),(#246035,#246036,#246037),(#246038,#246039,#246040),
(#246041,#246042,#246043)),.UNSPECIFIED.,.F.,.F.,.F.)
B_SPLINE_SURFACE_WITH_KNOTS((4,2,4),(3,3),(0.,0.000257953807872843,0.000515907615745687),
(0.,1.),.UNSPECIFIED.)
GEOMETRIC_REPRESENTATION_ITEM()
RATIONAL_B_SPLINE_SURFACE(((1.,0.87461970713939,1.),(1.,0.874834349679608,
1.),(1.,0.854686104156984,1.),(1.,0.792476597915946,1.),(1.,0.750887854594552,
1.),(1.,0.705585838031425,1.)))
REPRESENTATION_ITEM('')
SURFACE()
);
#3530=(
BOUNDED_SURFACE()
B_SPLINE_SURFACE(3,2,((#246049,#246050,#246051),(#246052,#246053,#246054),
(#246055,#246056,#246057),(#246058,#246059,#246060)),.UNSPECIFIED.,.F.,
 .F.,.F.)
B_SPLINE_SURFACE_WITH_KNOTS((4,4),(3,3),(0.,0.000511815437699149),(0.,1.00105881331542),
 .UNSPECIFIED.)
GEOMETRIC_REPRESENTATION_ITEM()
RATIONAL_B_SPLINE_SURFACE(((1.,0.706796661946474,1.00062089519691),(1.,
0.707430821225348,1.00061955228434),(1.,0.708058545830872,1.00061822299799),
(1.,0.708394505252856,1.00061751156138)))
REPRESENTATION_ITEM('')
SURFACE()
);
#3531=(
BOUNDED_SURFACE()
B_SPLINE_SURFACE(3,2,((#246062,#246063,#246064),(#246065,#246066,#246067),
(#246068,#246069,#246070),(#246071,#246072,#246073),(#246074,#246075,#246076),
(#246077,#246078,#246079)),.UNSPECIFIED.,.F.,.F.,.F.)
B_SPLINE_SURFACE_WITH_KNOTS((4,2,4),(3,3),(0.,0.000256915317531268,0.000513830635062537),
(0.,1.),.UNSPECIFIED.)
GEOMETRIC_REPRESENTATION_ITEM()
RATIONAL_B_SPLINE_SURFACE(((1.,0.705585838031453,1.),(1.,0.75090243354269,
1.),(1.,0.792329530082585,1.),(1.,0.85428840159416,1.),(1.,0.874998031125199,
1.),(1.,0.874619707139421,1.)))
REPRESENTATION_ITEM('')
SURFACE()
);
#3532=(
BOUNDED_SURFACE()
B_SPLINE_SURFACE(3,2,((#246085,#246086,#246087),(#246088,#246089,#246090),
(#246091,#246092,#246093),(#246094,#246095,#246096),(#246097,#246098,#246099),
(#246100,#246101,#246102)),.UNSPECIFIED.,.F.,.F.,.F.)
B_SPLINE_SURFACE_WITH_KNOTS((4,2,4),(3,3),(-1.40946282423116E-17,0.000256592814262149,
0.000513185628524313),(0.,1.),.UNSPECIFIED.)
GEOMETRIC_REPRESENTATION_ITEM()
RATIONAL_B_SPLINE_SURFACE(((1.,0.708712527163669,1.),(1.,0.753780902613169,
1.),(1.,0.794538995769778,1.),(1.,0.855070770330537,1.),(1.,0.875018427445752,
1.),(1.,0.874619707139392,1.)))
REPRESENTATION_ITEM('')
SURFACE()
);
#3533=(
BOUNDED_SURFACE()
B_SPLINE_SURFACE(3,2,((#246104,#246105,#246106),(#246107,#246108,#246109),
(#246110,#246111,#246112),(#246113,#246114,#246115)),.UNSPECIFIED.,.F.,
 .F.,.F.)
B_SPLINE_SURFACE_WITH_KNOTS((4,4),(3,3),(0.,0.000511815072430413),(0.,1.00105598365874),
 .UNSPECIFIED.)
GEOMETRIC_REPRESENTATION_ITEM()
RATIONAL_B_SPLINE_SURFACE(((1.,0.706797490733722,1.00061923411697),(1.,
0.706182062146645,1.00062053388204),(1.,0.705584062768979,1.00062179683718),
(1.,0.705266224770506,1.00062246810064)))
REPRESENTATION_ITEM('')
SURFACE()
);
#3534=(
BOUNDED_SURFACE()
B_SPLINE_SURFACE(3,2,((#246121,#246122,#246123),(#246124,#246125,#246126),
(#246127,#246128,#246129),(#246130,#246131,#246132),(#246133,#246134,#246135),
(#246136,#246137,#246138)),.UNSPECIFIED.,.F.,.F.,.F.)
B_SPLINE_SURFACE_WITH_KNOTS((4,2,4),(3,3),(0.,0.000257652232350891,0.000515304464701781),
(0.,1.),.UNSPECIFIED.)
GEOMETRIC_REPRESENTATION_ITEM()
RATIONAL_B_SPLINE_SURFACE(((1.,0.874619707139378,1.),(1.,0.87486118043044,
1.),(1.,0.85545572592119,1.),(1.,0.794699358954915,1.),(1.,0.75376897778887,
1.),(1.,0.708712527163644,1.)))
REPRESENTATION_ITEM('')
SURFACE()
);
#3535=(
BOUNDED_SURFACE()
B_SPLINE_SURFACE(3,2,((#246144,#246145,#246146),(#246147,#246148,#246149),
(#246150,#246151,#246152),(#246153,#246154,#246155)),.UNSPECIFIED.,.F.,
 .F.,.F.)
B_SPLINE_SURFACE_WITH_KNOTS((4,4),(3,3),(-5.42101086242752E-20,0.000397394373651921),
(0.,1.),.UNSPECIFIED.)
GEOMETRIC_REPRESENTATION_ITEM()
RATIONAL_B_SPLINE_SURFACE(((1.,0.707106781186562,1.),(1.,0.707752587915892,
1.),(1.,0.708377654540671,1.),(1.,0.708689770883324,1.)))
REPRESENTATION_ITEM('')
SURFACE()
);
#3536=(
BOUNDED_SURFACE()
B_SPLINE_SURFACE(3,2,((#246157,#246158,#246159),(#246160,#246161,#246162),
(#246163,#246164,#246165),(#246166,#246167,#246168)),.UNSPECIFIED.,.F.,
 .F.,.F.)
B_SPLINE_SURFACE_WITH_KNOTS((4,4),(3,3),(-5.63785129692462E-18,0.000511815456479789),
(0.,1.00105873159701),.UNSPECIFIED.)
GEOMETRIC_REPRESENTATION_ITEM()
RATIONAL_B_SPLINE_SURFACE(((1.,0.708394529057188,1.0006174638519),(1.,0.708058564167717,
1.00061817524519),(1.,0.70743083537295,1.0006195044378),(1.,0.706796685881218,
1.00062084722601)))
REPRESENTATION_ITEM('')
SURFACE()
);
#3537=(
BOUNDED_SURFACE()
B_SPLINE_SURFACE(3,2,((#246174,#246175,#246176),(#246177,#246178,#246179),
(#246180,#246181,#246182),(#246183,#246184,#246185)),.UNSPECIFIED.,.F.,
 .F.,.F.)
B_SPLINE_SURFACE_WITH_KNOTS((4,4),(3,3),(-1.38777878078145E-17,0.000397394465448301),
(0.,1.),.UNSPECIFIED.)
GEOMETRIC_REPRESENTATION_ITEM()
RATIONAL_B_SPLINE_SURFACE(((1.,0.705498956110756,1.),(1.,0.705821764811832,
1.),(1.,0.706461952521107,1.),(1.,0.707106781186571,1.)))
REPRESENTATION_ITEM('')
SURFACE()
);
#3538=(
BOUNDED_SURFACE()
B_SPLINE_SURFACE(3,2,((#246191,#246192,#246193),(#246194,#246195,#246196),
(#246197,#246198,#246199),(#246200,#246201,#246202)),.UNSPECIFIED.,.F.,
 .F.,.F.)
B_SPLINE_SURFACE_WITH_KNOTS((4,4),(3,3),(-4.87890977618477E-19,0.000397394410828747),
(0.,1.),.UNSPECIFIED.)
GEOMETRIC_REPRESENTATION_ITEM()
RATIONAL_B_SPLINE_SURFACE(((1.,0.708689770883332,1.),(1.,0.708376440034503,
1.),(1.,0.707750498698384,1.),(1.,0.707106781186558,1.)))
REPRESENTATION_ITEM('')
SURFACE()
);
#3539=(
BOUNDED_SURFACE()
B_SPLINE_SURFACE(3,2,((#246208,#246209,#246210),(#246211,#246212,#246213),
(#246214,#246215,#246216),(#246217,#246218,#246219)),.UNSPECIFIED.,.F.,
 .F.,.F.)
B_SPLINE_SURFACE_WITH_KNOTS((4,4),(3,3),(0.,0.000511815090126181),(0.,1.00105592270224),
 .UNSPECIFIED.)
GEOMETRIC_REPRESENTATION_ITEM()
RATIONAL_B_SPLINE_SURFACE(((1.,0.705266242717473,1.00062243213086),(1.,
0.705584085909101,1.00062176089518),(1.,0.706182089450503,1.00062049800415),
(1.,0.706797508587471,1.00061919833407)))
REPRESENTATION_ITEM('')
SURFACE()
);
#3540=(
BOUNDED_SURFACE()
B_SPLINE_SURFACE(3,2,((#246221,#246222,#246223),(#246224,#246225,#246226),
(#246227,#246228,#246229),(#246230,#246231,#246232)),.UNSPECIFIED.,.F.,
 .F.,.F.)
B_SPLINE_SURFACE_WITH_KNOTS((4,4),(3,3),(0.,0.000397394428086631),(0.,1.),
 .UNSPECIFIED.)
GEOMETRIC_REPRESENTATION_ITEM()
RATIONAL_B_SPLINE_SURFACE(((1.,0.70710678118655,1.),(1.,0.706459846759093,
1.),(1.,0.705820510737295,1.),(1.,0.705498956110744,1.)))
REPRESENTATION_ITEM('')
SURFACE()
);
#3541=(
BOUNDED_SURFACE()
B_SPLINE_SURFACE(3,2,((#246238,#246239,#246240),(#246241,#246242,#246243),
(#246244,#246245,#246246),(#246247,#246248,#246249),(#246250,#246251,#246252),
(#246253,#246254,#246255)),.UNSPECIFIED.,.F.,.F.,.F.)
B_SPLINE_SURFACE_WITH_KNOTS((4,2,4),(3,3),(0.,0.000257953807872851,0.000515907615745702),
(0.,1.),.UNSPECIFIED.)
GEOMETRIC_REPRESENTATION_ITEM()
RATIONAL_B_SPLINE_SURFACE(((1.,0.874619707139391,1.),(1.,0.874834349679692,
1.),(1.,0.85468610415687,1.),(1.,0.792476597916061,1.),(1.,0.750887854594425,
1.),(1.,0.705585838031435,1.)))
REPRESENTATION_ITEM('')
SURFACE()
);
#3542=(
BOUNDED_SURFACE()
B_SPLINE_SURFACE(3,2,((#246261,#246262,#246263),(#246264,#246265,#246266),
(#246267,#246268,#246269),(#246270,#246271,#246272)),.UNSPECIFIED.,.F.,
 .F.,.F.)
B_SPLINE_SURFACE_WITH_KNOTS((4,4),(3,3),(0.,0.000511815437699153),(0.,1.00105881331651),
 .UNSPECIFIED.)
GEOMETRIC_REPRESENTATION_ITEM()
RATIONAL_B_SPLINE_SURFACE(((1.,0.706796661946155,1.00062089519755),(1.,
0.707430821225017,1.00061955228497),(1.,0.708058545830544,1.00061822299863),
(1.,0.708394505252542,1.00061751156201)))
REPRESENTATION_ITEM('')
SURFACE()
);
#3543=(
BOUNDED_SURFACE()
B_SPLINE_SURFACE(3,2,((#246274,#246275,#246276),(#246277,#246278,#246279),
(#246280,#246281,#246282),(#246283,#246284,#246285),(#246286,#246287,#246288),
(#246289,#246290,#246291)),.UNSPECIFIED.,.F.,.F.,.F.)
B_SPLINE_SURFACE_WITH_KNOTS((4,2,4),(3,3),(1.35525271560688E-18,0.000256915317531269,
0.000513830635062536),(0.,1.),.UNSPECIFIED.)
GEOMETRIC_REPRESENTATION_ITEM()
RATIONAL_B_SPLINE_SURFACE(((1.,0.705585838031444,1.),(1.,0.750902433542528,
1.),(1.,0.792329530082818,1.),(1.,0.854288401593931,1.),(1.,0.87499803112536,
1.),(1.,0.874619707139404,1.)))
REPRESENTATION_ITEM('')
SURFACE()
);
#3544=(
BOUNDED_SURFACE()
B_SPLINE_SURFACE(3,2,((#246297,#246298,#246299),(#246300,#246301,#246302),
(#246303,#246304,#246305),(#246306,#246307,#246308),(#246309,#246310,#246311),
(#246312,#246313,#246314)),.UNSPECIFIED.,.F.,.F.,.F.)
B_SPLINE_SURFACE_WITH_KNOTS((4,2,4),(3,3),(-1.33627917758838E-17,0.000256592814262148,
0.00051318562852431),(0.,1.),.UNSPECIFIED.)
GEOMETRIC_REPRESENTATION_ITEM()
RATIONAL_B_SPLINE_SURFACE(((1.,0.708712527163659,1.),(1.,0.753780902613647,
1.),(1.,0.794538995769118,1.),(1.,0.855070770331176,1.),(1.,0.875018427445279,
1.),(1.,0.874619707139401,1.)))
REPRESENTATION_ITEM('')
SURFACE()
);
#3545=(
BOUNDED_SURFACE()
B_SPLINE_SURFACE(3,2,((#246316,#246317,#246318),(#246319,#246320,#246321),
(#246322,#246323,#246324),(#246325,#246326,#246327)),.UNSPECIFIED.,.F.,
 .F.,.F.)
B_SPLINE_SURFACE_WITH_KNOTS((4,4),(3,3),(0.,0.000511815072430395),(0.,1.00105598365649),
 .UNSPECIFIED.)
GEOMETRIC_REPRESENTATION_ITEM()
RATIONAL_B_SPLINE_SURFACE(((1.,0.706797490734372,1.00061923411566),(1.,
0.706182062147344,1.00062053388071),(1.,0.705584062769602,1.00062179683585),
(1.,0.705266224771175,1.00062246809932)))
REPRESENTATION_ITEM('')
SURFACE()
);
#3546=(
BOUNDED_SURFACE()
B_SPLINE_SURFACE(3,2,((#246333,#246334,#246335),(#246336,#246337,#246338),
(#246339,#246340,#246341),(#246342,#246343,#246344),(#246345,#246346,#246347),
(#246348,#246349,#246350)),.UNSPECIFIED.,.F.,.F.,.F.)
B_SPLINE_SURFACE_WITH_KNOTS((4,2,4),(3,3),(0.,0.000257652232350881,0.000515304464701762),
(0.,1.),.UNSPECIFIED.)
GEOMETRIC_REPRESENTATION_ITEM()
RATIONAL_B_SPLINE_SURFACE(((1.,0.874619707139381,1.),(1.,0.874861180430671,
1.),(1.,0.855455725920884,1.),(1.,0.794699358955244,1.),(1.,0.75376897778864,
1.),(1.,0.708712527163656,1.)))
REPRESENTATION_ITEM('')
SURFACE()
);
#3547=(
BOUNDED_SURFACE()
B_SPLINE_SURFACE(3,2,((#246356,#246357,#246358),(#246359,#246360,#246361),
(#246362,#246363,#246364),(#246365,#246366,#246367)),.UNSPECIFIED.,.F.,
 .F.,.F.)
B_SPLINE_SURFACE_WITH_KNOTS((4,4),(3,3),(0.,0.000397394373651913),(0.,1.),
 .UNSPECIFIED.)
GEOMETRIC_REPRESENTATION_ITEM()
RATIONAL_B_SPLINE_SURFACE(((1.,0.707106781186537,1.),(1.,0.707752587915933,
1.),(1.,0.708377654540649,1.),(1.,0.708689770883327,1.)))
REPRESENTATION_ITEM('')
SURFACE()
);
#3548=(
BOUNDED_SURFACE()
B_SPLINE_SURFACE(3,2,((#246369,#246370,#246371),(#246372,#246373,#246374),
(#246375,#246376,#246377),(#246378,#246379,#246380)),.UNSPECIFIED.,.F.,
 .F.,.F.)
B_SPLINE_SURFACE_WITH_KNOTS((4,4),(3,3),(0.,0.000511815456479784),(0.,1.00105873159913),
 .UNSPECIFIED.)
GEOMETRIC_REPRESENTATION_ITEM()
RATIONAL_B_SPLINE_SURFACE(((1.,0.708394529056561,1.00061746385314),(1.,
0.708058564167131,1.00061817524643),(1.,0.707430835372305,1.00061950443905),
(1.,0.706796685880607,1.00062084722726)))
REPRESENTATION_ITEM('')
SURFACE()
);
#3549=(
BOUNDED_SURFACE()
B_SPLINE_SURFACE(3,2,((#246386,#246387,#246388),(#246389,#246390,#246391),
(#246392,#246393,#246394),(#246395,#246396,#246397)),.UNSPECIFIED.,.F.,
 .F.,.F.)
B_SPLINE_SURFACE_WITH_KNOTS((4,4),(3,3),(8.13151629364128E-20,0.000397394465448307),
(0.,1.),.UNSPECIFIED.)
GEOMETRIC_REPRESENTATION_ITEM()
RATIONAL_B_SPLINE_SURFACE(((1.,0.70549895611076,1.),(1.,0.7058217648118,
1.),(1.,0.706461952521123,1.),(1.,0.707106781186563,1.)))
REPRESENTATION_ITEM('')
SURFACE()
);
#3550=(
BOUNDED_SURFACE()
B_SPLINE_SURFACE(3,2,((#246403,#246404,#246405),(#246406,#246407,#246408),
(#246409,#246410,#246411),(#246412,#246413,#246414)),.UNSPECIFIED.,.F.,
 .F.,.F.)
B_SPLINE_SURFACE_WITH_KNOTS((4,4),(3,3),(-3.79470760369927E-19,0.000397394410828737),
(0.,1.),.UNSPECIFIED.)
GEOMETRIC_REPRESENTATION_ITEM()
RATIONAL_B_SPLINE_SURFACE(((1.,0.708689770883314,1.),(1.,0.708376440034537,
1.),(1.,0.707750498698401,1.),(1.,0.70710678118655,1.)))
REPRESENTATION_ITEM('')
SURFACE()
);
#3551=(
BOUNDED_SURFACE()
B_SPLINE_SURFACE(3,2,((#246420,#246421,#246422),(#246423,#246424,#246425),
(#246426,#246427,#246428),(#246429,#246430,#246431)),.UNSPECIFIED.,.F.,
 .F.,.F.)
B_SPLINE_SURFACE_WITH_KNOTS((4,4),(3,3),(0.,0.000511815090126176),(0.,1.00105592270117),
 .UNSPECIFIED.)
GEOMETRIC_REPRESENTATION_ITEM()
RATIONAL_B_SPLINE_SURFACE(((1.,0.705266242717781,1.00062243213023),(1.,
0.705584085909421,1.00062176089455),(1.,0.706182089450807,1.00062049800352),
(1.,0.706797508587779,1.00061919833345)))
REPRESENTATION_ITEM('')
SURFACE()
);
#3552=(
BOUNDED_SURFACE()
B_SPLINE_SURFACE(3,2,((#246433,#246434,#246435),(#246436,#246437,#246438),
(#246439,#246440,#246441),(#246442,#246443,#246444)),.UNSPECIFIED.,.F.,
 .F.,.F.)
B_SPLINE_SURFACE_WITH_KNOTS((4,4),(3,3),(0.,0.000397394428086637),(0.,1.),
 .UNSPECIFIED.)
GEOMETRIC_REPRESENTATION_ITEM()
RATIONAL_B_SPLINE_SURFACE(((1.,0.707106781186535,1.),(1.,0.706459846759099,
1.),(1.,0.705820510737271,1.),(1.,0.705498956110739,1.)))
REPRESENTATION_ITEM('')
SURFACE()
);
#3553=(
BOUNDED_SURFACE()
B_SPLINE_SURFACE(3,2,((#246450,#246451,#246452),(#246453,#246454,#246455),
(#246456,#246457,#246458),(#246459,#246460,#246461),(#246462,#246463,#246464),
(#246465,#246466,#246467)),.UNSPECIFIED.,.F.,.F.,.F.)
B_SPLINE_SURFACE_WITH_KNOTS((4,2,4),(3,3),(0.,0.000257953807872846,0.000515907615745692),
(0.,1.),.UNSPECIFIED.)
GEOMETRIC_REPRESENTATION_ITEM()
RATIONAL_B_SPLINE_SURFACE(((1.,0.874619707139395,1.),(1.,0.874834349679225,
1.),(1.,0.854686104157495,1.),(1.,0.792476597915437,1.),(1.,0.750887854594915,
1.),(1.,0.705585838031433,1.)))
REPRESENTATION_ITEM('')
SURFACE()
);
#3554=(
BOUNDED_SURFACE()
B_SPLINE_SURFACE(3,2,((#246473,#246474,#246475),(#246476,#246477,#246478),
(#246479,#246480,#246481),(#246482,#246483,#246484)),.UNSPECIFIED.,.F.,
 .F.,.F.)
B_SPLINE_SURFACE_WITH_KNOTS((4,4),(3,3),(0.,0.00051181543769915),(0.,1.00105881331661),
 .UNSPECIFIED.)
GEOMETRIC_REPRESENTATION_ITEM()
RATIONAL_B_SPLINE_SURFACE(((1.,0.706796661946118,1.00062089519761),(1.,
0.707430821224989,1.00061955228504),(1.,0.708058545830539,1.00061822299869),
(1.,0.708394505252492,1.00061751156207)))
REPRESENTATION_ITEM('')
SURFACE()
);
#3555=(
BOUNDED_SURFACE()
B_SPLINE_SURFACE(3,2,((#246486,#246487,#246488),(#246489,#246490,#246491),
(#246492,#246493,#246494),(#246495,#246496,#246497),(#246498,#246499,#246500),
(#246501,#246502,#246503)),.UNSPECIFIED.,.F.,.F.,.F.)
B_SPLINE_SURFACE_WITH_KNOTS((4,2,4),(3,3),(1.19262238973405E-18,0.000256915317531265,
0.000513830635062528),(0.,1.),.UNSPECIFIED.)
GEOMETRIC_REPRESENTATION_ITEM()
RATIONAL_B_SPLINE_SURFACE(((1.,0.705585838031449,1.),(1.,0.750902433542299,
1.),(1.,0.792329530083107,1.),(1.,0.854288401593629,1.),(1.,0.874998031125559,
1.),(1.,0.874619707139395,1.)))
REPRESENTATION_ITEM('')
SURFACE()
);
#3556=(
BOUNDED_SURFACE()
B_SPLINE_SURFACE(3,2,((#246509,#246510,#246511),(#246512,#246513,#246514),
(#246515,#246516,#246517),(#246518,#246519,#246520),(#246521,#246522,#246523),
(#246524,#246525,#246526)),.UNSPECIFIED.,.F.,.F.,.F.)
B_SPLINE_SURFACE_WITH_KNOTS((4,2,4),(3,3),(-4.41812385287843E-18,0.000256592814262153,
0.00051318562852431),(0.,1.),.UNSPECIFIED.)
GEOMETRIC_REPRESENTATION_ITEM()
RATIONAL_B_SPLINE_SURFACE(((1.,0.708712527163687,1.),(1.,0.753780902613256,
1.),(1.,0.79453899576962,1.),(1.,0.855070770330703,1.),(1.,0.875018427445644,
1.),(1.,0.874619707139394,1.)))
REPRESENTATION_ITEM('')
SURFACE()
);
#3557=(
BOUNDED_SURFACE()
B_SPLINE_SURFACE(3,2,((#246528,#246529,#246530),(#246531,#246532,#246533),
(#246534,#246535,#246536),(#246537,#246538,#246539)),.UNSPECIFIED.,.F.,
 .F.,.F.)
B_SPLINE_SURFACE_WITH_KNOTS((4,4),(3,3),(-6.64073830647371E-18,0.000511815072430408),
(0.,1.00105598365564),.UNSPECIFIED.)
GEOMETRIC_REPRESENTATION_ITEM()
RATIONAL_B_SPLINE_SURFACE(((1.,0.70679749073463,1.00061923411516),(1.,0.706182062147569,
1.00062053388021),(1.,0.705584062769927,1.00062179683535),(1.,0.70526622477141,
1.00062246809881)))
REPRESENTATION_ITEM('')
SURFACE()
);
#3558=(
BOUNDED_SURFACE()
B_SPLINE_SURFACE(3,2,((#246545,#246546,#246547),(#246548,#246549,#246550),
(#246551,#246552,#246553),(#246554,#246555,#246556),(#246557,#246558,#246559),
(#246560,#246561,#246562)),.UNSPECIFIED.,.F.,.F.,.F.)
B_SPLINE_SURFACE_WITH_KNOTS((4,2,4),(3,3),(0.,0.00025765223235088,0.00051530446470176),
(0.,1.),.UNSPECIFIED.)
GEOMETRIC_REPRESENTATION_ITEM()
RATIONAL_B_SPLINE_SURFACE(((1.,0.874619707139391,1.),(1.,0.874861180429929,
1.),(1.,0.85545572592193,1.),(1.,0.794699358954205,1.),(1.,0.753768977789438,
1.),(1.,0.708712527163671,1.)))
REPRESENTATION_ITEM('')
SURFACE()
);
#3559=(
BOUNDED_SURFACE()
B_SPLINE_SURFACE(3,2,((#246568,#246569,#246570),(#246571,#246572,#246573),
(#246574,#246575,#246576),(#246577,#246578,#246579)),.UNSPECIFIED.,.F.,
 .F.,.F.)
B_SPLINE_SURFACE_WITH_KNOTS((4,4),(3,3),(-6.64073830647371E-18,0.000397394373651924),
(0.,1.),.UNSPECIFIED.)
GEOMETRIC_REPRESENTATION_ITEM()
RATIONAL_B_SPLINE_SURFACE(((1.,0.707106781186545,1.),(1.,0.707752587915891,
1.),(1.,0.708377654540681,1.),(1.,0.708689770883316,1.)))
REPRESENTATION_ITEM('')
SURFACE()
);
#3560=(
BOUNDED_SURFACE()
B_SPLINE_SURFACE(3,2,((#246581,#246582,#246583),(#246584,#246585,#246586),
(#246587,#246588,#246589),(#246590,#246591,#246592)),.UNSPECIFIED.,.F.,
 .F.,.F.)
B_SPLINE_SURFACE_WITH_KNOTS((4,4),(3,3),(3.22550146314438E-18,0.000511815456479793),
(0.,1.00105873160129),.UNSPECIFIED.)
GEOMETRIC_REPRESENTATION_ITEM()
RATIONAL_B_SPLINE_SURFACE(((1.,0.708394529055928,1.0006174638544),(1.,0.708058564166499,
1.00061817524769),(1.,0.707430835371648,1.00061950444031),(1.,0.706796685879989,
1.00062084722853)))
REPRESENTATION_ITEM('')
SURFACE()
);
#3561=(
BOUNDED_SURFACE()
B_SPLINE_SURFACE(3,2,((#246598,#246599,#246600),(#246601,#246602,#246603),
(#246604,#246605,#246606),(#246607,#246608,#246609)),.UNSPECIFIED.,.F.,
 .F.,.F.)
B_SPLINE_SURFACE_WITH_KNOTS((4,4),(3,3),(-6.96599895821937E-18,0.000397394465448294),
(0.,1.),.UNSPECIFIED.)
GEOMETRIC_REPRESENTATION_ITEM()
RATIONAL_B_SPLINE_SURFACE(((1.,0.705498956110761,1.),(1.,0.705821764811777,
1.),(1.,0.706461952521158,1.),(1.,0.707106781186545,1.)))
REPRESENTATION_ITEM('')
SURFACE()
);
#3562=(
BOUNDED_SURFACE()
B_SPLINE_SURFACE(3,2,((#246615,#246616,#246617),(#246618,#246619,#246620),
(#246621,#246622,#246623),(#246624,#246625,#246626)),.UNSPECIFIED.,.F.,
 .F.,.F.)
B_SPLINE_SURFACE_WITH_KNOTS((4,4),(3,3),(0.,0.000397394410828746),(0.,1.),
 .UNSPECIFIED.)
GEOMETRIC_REPRESENTATION_ITEM()
RATIONAL_B_SPLINE_SURFACE(((1.,0.708689770883335,1.),(1.,0.708376440034449,
1.),(1.,0.70775049869843,1.),(1.,0.707106781186545,1.)))
REPRESENTATION_ITEM('')
SURFACE()
);
#3563=(
BOUNDED_SURFACE()
B_SPLINE_SURFACE(3,2,((#246632,#246633,#246634),(#246635,#246636,#246637),
(#246638,#246639,#246640),(#246641,#246642,#246643)),.UNSPECIFIED.,.F.,
 .F.,.F.)
B_SPLINE_SURFACE_WITH_KNOTS((4,4),(3,3),(1.35525271560688E-19,0.000511815090126177),
(0.,1.00105592270336),.UNSPECIFIED.)
GEOMETRIC_REPRESENTATION_ITEM()
RATIONAL_B_SPLINE_SURFACE(((1.,0.705266242717142,1.00062243213152),(1.,
0.705584085908801,1.00062176089584),(1.,0.70618208945015,1.00062049800481),
(1.,0.706797508587144,1.00061919833473)))
REPRESENTATION_ITEM('')
SURFACE()
);
#3564=(
BOUNDED_SURFACE()
B_SPLINE_SURFACE(3,2,((#246645,#246646,#246647),(#246648,#246649,#246650),
(#246651,#246652,#246653),(#246654,#246655,#246656)),.UNSPECIFIED.,.F.,
 .F.,.F.)
B_SPLINE_SURFACE_WITH_KNOTS((4,4),(3,3),(-7.26415455565288E-18,0.000397394428086627),
(0.,1.),.UNSPECIFIED.)
GEOMETRIC_REPRESENTATION_ITEM()
RATIONAL_B_SPLINE_SURFACE(((1.,0.707106781186549,1.),(1.,0.70645984675907,
1.),(1.,0.705820510737295,1.),(1.,0.705498956110751,1.)))
REPRESENTATION_ITEM('')
SURFACE()
);
#3565=(
BOUNDED_SURFACE()
B_SPLINE_SURFACE(3,2,((#246662,#246663,#246664),(#246665,#246666,#246667),
(#246668,#246669,#246670),(#246671,#246672,#246673),(#246674,#246675,#246676),
(#246677,#246678,#246679)),.UNSPECIFIED.,.F.,.F.,.F.)
B_SPLINE_SURFACE_WITH_KNOTS((4,2,4),(3,3),(5.14996031930615E-19,0.000257953807872838,
0.000515907615745675),(0.,1.),.UNSPECIFIED.)
GEOMETRIC_REPRESENTATION_ITEM()
RATIONAL_B_SPLINE_SURFACE(((1.,0.874619707139394,1.),(1.,0.874834349678729,
1.),(1.,0.854686104158156,1.),(1.,0.792476597914813,1.),(1.,0.750887854595356,
1.),(1.,0.705585838031451,1.)))
REPRESENTATION_ITEM('')
SURFACE()
);
#3566=(
BOUNDED_SURFACE()
B_SPLINE_SURFACE(3,2,((#246685,#246686,#246687),(#246688,#246689,#246690),
(#246691,#246692,#246693),(#246694,#246695,#246696)),.UNSPECIFIED.,.F.,
 .F.,.F.)
B_SPLINE_SURFACE_WITH_KNOTS((4,4),(3,3),(0.,0.000511815437699148),(0.,1.00105881331611),
 .UNSPECIFIED.)
GEOMETRIC_REPRESENTATION_ITEM()
RATIONAL_B_SPLINE_SURFACE(((1.,0.706796661946273,1.00062089519732),(1.,
0.707430821225126,1.00061955228474),(1.,0.708058545830682,1.0006182229984),
(1.,0.708394505252651,1.00061751156178)))
REPRESENTATION_ITEM('')
SURFACE()
);
#3567=(
BOUNDED_SURFACE()
B_SPLINE_SURFACE(3,2,((#246698,#246699,#246700),(#246701,#246702,#246703),
(#246704,#246705,#246706),(#246707,#246708,#246709),(#246710,#246711,#246712),
(#246713,#246714,#246715)),.UNSPECIFIED.,.F.,.F.,.F.)
B_SPLINE_SURFACE_WITH_KNOTS((4,2,4),(3,3),(0.,0.00025691531753126,0.00051383063506252),
(0.,1.),.UNSPECIFIED.)
GEOMETRIC_REPRESENTATION_ITEM()
RATIONAL_B_SPLINE_SURFACE(((1.,0.705585838031466,1.),(1.,0.75090243354285,
1.),(1.,0.792329530082371,1.),(1.,0.854288401594364,1.),(1.,0.874998031125017,
1.),(1.,0.874619707139408,1.)))
REPRESENTATION_ITEM('')
SURFACE()
);
#3568=(
BOUNDED_SURFACE()
B_SPLINE_SURFACE(3,2,((#246721,#246722,#246723),(#246724,#246725,#246726),
(#246727,#246728,#246729),(#246730,#246731,#246732),(#246733,#246734,#246735),
(#246736,#246737,#246738)),.UNSPECIFIED.,.F.,.F.,.F.)
B_SPLINE_SURFACE_WITH_KNOTS((4,2,4),(3,3),(-1.07607065619186E-17,0.000256592814262151,
0.000513185628524313),(0.,1.),.UNSPECIFIED.)
GEOMETRIC_REPRESENTATION_ITEM()
RATIONAL_B_SPLINE_SURFACE(((1.,0.708712527163685,1.),(1.,0.753780902613632,
1.),(1.,0.794538995769127,1.),(1.,0.855070770331165,1.),(1.,0.875018427445278,
1.),(1.,0.874619707139394,1.)))
REPRESENTATION_ITEM('')
SURFACE()
);
#3569=(
BOUNDED_SURFACE()
B_SPLINE_SURFACE(3,2,((#246740,#246741,#246742),(#246743,#246744,#246745),
(#246746,#246747,#246748),(#246749,#246750,#246751)),.UNSPECIFIED.,.F.,
 .F.,.F.)
B_SPLINE_SURFACE_WITH_KNOTS((4,4),(3,3),(0.,0.000511815072430402),(0.,1.00105598365829),
 .UNSPECIFIED.)
GEOMETRIC_REPRESENTATION_ITEM()
RATIONAL_B_SPLINE_SURFACE(((1.,0.706797490733853,1.00061923411671),(1.,
0.70618206214678,1.00062053388177),(1.,0.705584062769139,1.00062179683691),
(1.,0.705266224770619,1.00062246810038)))
REPRESENTATION_ITEM('')
SURFACE()
);
#3570=(
BOUNDED_SURFACE()
B_SPLINE_SURFACE(3,2,((#246757,#246758,#246759),(#246760,#246761,#246762),
(#246763,#246764,#246765),(#246766,#246767,#246768),(#246769,#246770,#246771),
(#246772,#246773,#246774)),.UNSPECIFIED.,.F.,.F.,.F.)
B_SPLINE_SURFACE_WITH_KNOTS((4,2,4),(3,3),(0.,0.000257652232350876,0.000515304464701751),
(0.,1.),.UNSPECIFIED.)
GEOMETRIC_REPRESENTATION_ITEM()
RATIONAL_B_SPLINE_SURFACE(((1.,0.874619707139385,1.),(1.,0.874861180430971,
1.),(1.,0.855455725920496,1.),(1.,0.794699358955617,1.),(1.,0.753768977788383,
1.),(1.,0.708712527163647,1.)))
REPRESENTATION_ITEM('')
SURFACE()
);
#3571=(
BOUNDED_SURFACE()
B_SPLINE_SURFACE(3,2,((#246780,#246781,#246782),(#246783,#246784,#246785),
(#246786,#246787,#246788),(#246789,#246790,#246791)),.UNSPECIFIED.,.F.,
 .F.,.F.)
B_SPLINE_SURFACE_WITH_KNOTS((4,4),(3,3),(0.,0.000397394373651911),(0.,1.),
 .UNSPECIFIED.)
GEOMETRIC_REPRESENTATION_ITEM()
RATIONAL_B_SPLINE_SURFACE(((1.,0.707106781186554,1.),(1.,0.707752587915894,
1.),(1.,0.708377654540672,1.),(1.,0.708689770883338,1.)))
REPRESENTATION_ITEM('')
SURFACE()
);
#3572=(
BOUNDED_SURFACE()
B_SPLINE_SURFACE(3,2,((#246793,#246794,#246795),(#246796,#246797,#246798),
(#246799,#246800,#246801),(#246802,#246803,#246804)),.UNSPECIFIED.,.F.,
 .F.,.F.)
B_SPLINE_SURFACE_WITH_KNOTS((4,4),(3,3),(-2.54787510534094E-18,0.000511815456479783),
(0.,1.00105873160091),.UNSPECIFIED.)
GEOMETRIC_REPRESENTATION_ITEM()
RATIONAL_B_SPLINE_SURFACE(((1.,0.708394529056051,1.00061746385417),(1.,
0.708058564166611,1.00061817524746),(1.,0.707430835371771,1.00061950444008),
(1.,0.706796685880101,1.0006208472283)))
REPRESENTATION_ITEM('')
SURFACE()
);
#3573=(
BOUNDED_SURFACE()
B_SPLINE_SURFACE(3,2,((#246810,#246811,#246812),(#246813,#246814,#246815),
(#246816,#246817,#246818),(#246819,#246820,#246821)),.UNSPECIFIED.,.F.,
 .F.,.F.)
B_SPLINE_SURFACE_WITH_KNOTS((4,4),(3,3),(0.,0.00039739446544831),(0.,1.),
 .UNSPECIFIED.)
GEOMETRIC_REPRESENTATION_ITEM()
RATIONAL_B_SPLINE_SURFACE(((1.,0.70549895611077,1.),(1.,0.705821764811747,
1.),(1.,0.706461952521146,1.),(1.,0.707106781186554,1.)))
REPRESENTATION_ITEM('')
SURFACE()
);
#3574=(
BOUNDED_SURFACE()
B_SPLINE_SURFACE(3,2,((#246827,#246828,#246829),(#246830,#246831,#246832),
(#246833,#246834,#246835),(#246836,#246837,#246838)),.UNSPECIFIED.,.F.,
 .F.,.F.)
B_SPLINE_SURFACE_WITH_KNOTS((4,4),(3,3),(-2.71050543121376E-20,0.000397394410828737),
(0.,1.),.UNSPECIFIED.)
GEOMETRIC_REPRESENTATION_ITEM()
RATIONAL_B_SPLINE_SURFACE(((1.,0.708689770883326,1.),(1.,0.708376440034482,
1.),(1.,0.707750498698405,1.),(1.,0.707106781186548,1.)))
REPRESENTATION_ITEM('')
SURFACE()
);
#3575=(
BOUNDED_SURFACE()
B_SPLINE_SURFACE(3,2,((#246844,#246845,#246846),(#246847,#246848,#246849),
(#246850,#246851,#246852),(#246853,#246854,#246855)),.UNSPECIFIED.,.F.,
 .F.,.F.)
B_SPLINE_SURFACE_WITH_KNOTS((4,4),(3,3),(2.71050543121376E-20,0.000511815090126173),
(0.,1.00105592270303),.UNSPECIFIED.)
GEOMETRIC_REPRESENTATION_ITEM()
RATIONAL_B_SPLINE_SURFACE(((1.,0.705266242717242,1.00062243213133),(1.,
0.705584085908911,1.00062176089565),(1.,0.706182089450249,1.00062049800462),
(1.,0.70679750858724,1.00061919833454)))
REPRESENTATION_ITEM('')
SURFACE()
);
#3576=(
BOUNDED_SURFACE()
B_SPLINE_SURFACE(3,2,((#246857,#246858,#246859),(#246860,#246861,#246862),
(#246863,#246864,#246865),(#246866,#246867,#246868)),.UNSPECIFIED.,.F.,
 .F.,.F.)
B_SPLINE_SURFACE_WITH_KNOTS((4,4),(3,3),(-8.13151629364128E-20,0.000397394428086625),
(0.,1.),.UNSPECIFIED.)
GEOMETRIC_REPRESENTATION_ITEM()
RATIONAL_B_SPLINE_SURFACE(((1.,0.707106781186548,1.),(1.,0.706459846759093,
1.),(1.,0.70582051073728,1.),(1.,0.705498956110757,1.)))
REPRESENTATION_ITEM('')
SURFACE()
);
#3577=(
BOUNDED_SURFACE()
B_SPLINE_SURFACE(3,2,((#246874,#246875,#246876),(#246877,#246878,#246879),
(#246880,#246881,#246882),(#246883,#246884,#246885),(#246886,#246887,#246888),
(#246889,#246890,#246891)),.UNSPECIFIED.,.F.,.F.,.F.)
B_SPLINE_SURFACE_WITH_KNOTS((4,2,4),(3,3),(0.,0.00025795380787285,0.000515907615745701),
(0.,1.),.UNSPECIFIED.)
GEOMETRIC_REPRESENTATION_ITEM()
RATIONAL_B_SPLINE_SURFACE(((1.,0.874619707139389,1.),(1.,0.874834349678911,
1.),(1.,0.854686104157886,1.),(1.,0.792476597915053,1.),(1.,0.750887854595184,
1.),(1.,0.705585838031474,1.)))
REPRESENTATION_ITEM('')
SURFACE()
);
#3578=(
BOUNDED_SURFACE()
B_SPLINE_SURFACE(3,2,((#246897,#246898,#246899),(#246900,#246901,#246902),
(#246903,#246904,#246905),(#246906,#246907,#246908)),.UNSPECIFIED.,.F.,
 .F.,.F.)
B_SPLINE_SURFACE_WITH_KNOTS((4,4),(3,3),(-7.04731412115578E-18,0.000511815437699152),
(0.,1.00105881331506),.UNSPECIFIED.)
GEOMETRIC_REPRESENTATION_ITEM()
RATIONAL_B_SPLINE_SURFACE(((1.,0.706796661946578,1.0006208951967),(1.,0.707430821225437,
1.00061955228412),(1.,0.708058545830975,1.00061822299778),(1.,0.708394505252952,
1.00061751156116)))
REPRESENTATION_ITEM('')
SURFACE()
);
#3579=(
BOUNDED_SURFACE()
B_SPLINE_SURFACE(3,2,((#246910,#246911,#246912),(#246913,#246914,#246915),
(#246916,#246917,#246918),(#246919,#246920,#246921),(#246922,#246923,#246924),
(#246925,#246926,#246927)),.UNSPECIFIED.,.F.,.F.,.F.)
B_SPLINE_SURFACE_WITH_KNOTS((4,2,4),(3,3),(1.89735380184963E-19,0.000256915317531257,
0.000513830635062515),(0.,1.),.UNSPECIFIED.)
GEOMETRIC_REPRESENTATION_ITEM()
RATIONAL_B_SPLINE_SURFACE(((1.,0.705585838031421,1.),(1.,0.750902433543199,
1.),(1.,0.792329530081917,1.),(1.,0.854288401594789,1.),(1.,0.874998031124692,
1.),(1.,0.87461970713939,1.)))
REPRESENTATION_ITEM('')
SURFACE()
);
#3580=(
BOUNDED_SURFACE()
B_SPLINE_SURFACE(3,2,((#246933,#246934,#246935),(#246936,#246937,#246938),
(#246939,#246940,#246941),(#246942,#246943,#246944),(#246945,#246946,#246947),
(#246948,#246949,#246950)),.UNSPECIFIED.,.F.,.F.,.F.)
B_SPLINE_SURFACE_WITH_KNOTS((4,2,4),(3,3),(-1.07878116162308E-17,0.000256592814262151,
0.000513185628524312),(0.,1.),.UNSPECIFIED.)
GEOMETRIC_REPRESENTATION_ITEM()
RATIONAL_B_SPLINE_SURFACE(((1.,0.708712527163674,1.),(1.,0.753780902612964,
1.),(1.,0.794538995770014,1.),(1.,0.855070770330296,1.),(1.,0.875018427445928,
1.),(1.,0.874619707139402,1.)))
REPRESENTATION_ITEM('')
SURFACE()
);
#3581=(
BOUNDED_SURFACE()
B_SPLINE_SURFACE(3,2,((#246952,#246953,#246954),(#246955,#246956,#246957),
(#246958,#246959,#246960),(#246961,#246962,#246963)),.UNSPECIFIED.,.F.,
 .F.,.F.)
B_SPLINE_SURFACE_WITH_KNOTS((4,4),(3,3),(4.87890977618477E-19,0.000511815072430404),
(0.,1.00105598365881),.UNSPECIFIED.)
GEOMETRIC_REPRESENTATION_ITEM()
RATIONAL_B_SPLINE_SURFACE(((1.,0.706797490733706,1.00061923411701),(1.,
0.706182062146592,1.00062053388208),(1.,0.705584062769001,1.00062179683722),
(1.,0.70526622477046,1.00062246810068)))
REPRESENTATION_ITEM('')
SURFACE()
);
#3582=(
BOUNDED_SURFACE()
B_SPLINE_SURFACE(3,2,((#246969,#246970,#246971),(#246972,#246973,#246974),
(#246975,#246976,#246977),(#246978,#246979,#246980),(#246981,#246982,#246983),
(#246984,#246985,#246986)),.UNSPECIFIED.,.F.,.F.,.F.)
B_SPLINE_SURFACE_WITH_KNOTS((4,2,4),(3,3),(-2.24971950790742E-18,0.000257652232350876,
0.000515304464701754),(0.,1.),.UNSPECIFIED.)
GEOMETRIC_REPRESENTATION_ITEM()
RATIONAL_B_SPLINE_SURFACE(((1.,0.874619707139394,1.),(1.,0.874861180430937,
1.),(1.,0.855455725920569,1.),(1.,0.794699358955574,1.),(1.,0.753768977788433,
1.),(1.,0.708712527163671,1.)))
REPRESENTATION_ITEM('')
SURFACE()
);
#3583=(
BOUNDED_SURFACE()
B_SPLINE_SURFACE(3,2,((#246992,#246993,#246994),(#246995,#246996,#246997),
(#246998,#246999,#247000),(#247001,#247002,#247003)),.UNSPECIFIED.,.F.,
 .F.,.F.)
B_SPLINE_SURFACE_WITH_KNOTS((4,4),(3,3),(1.0842021724855E-19,0.000397394373651918),
(0.,1.),.UNSPECIFIED.)
GEOMETRIC_REPRESENTATION_ITEM()
RATIONAL_B_SPLINE_SURFACE(((1.,0.707106781186548,1.),(1.,0.707752587915899,
1.),(1.,0.708377654540685,1.),(1.,0.708689770883336,1.)))
REPRESENTATION_ITEM('')
SURFACE()
);
#3584=(
BOUNDED_SURFACE()
B_SPLINE_SURFACE(3,2,((#247005,#247006,#247007),(#247008,#247009,#247010),
(#247011,#247012,#247013),(#247014,#247015,#247016)),.UNSPECIFIED.,.F.,
 .F.,.F.)
B_SPLINE_SURFACE_WITH_KNOTS((4,4),(3,3),(-2.43945488809238E-18,0.000511815456479785),
(0.,1.00105873160026),.UNSPECIFIED.)
GEOMETRIC_REPRESENTATION_ITEM()
RATIONAL_B_SPLINE_SURFACE(((1.,0.708394529056247,1.00061746385379),(1.,
0.708058564166769,1.00061817524708),(1.,0.707430835371989,1.00061950443971),
(1.,0.706796685880284,1.00062084722792)))
REPRESENTATION_ITEM('')
SURFACE()
);
#3585=(
BOUNDED_SURFACE()
B_SPLINE_SURFACE(3,2,((#247022,#247023,#247024),(#247025,#247026,#247027),
(#247028,#247029,#247030),(#247031,#247032,#247033)),.UNSPECIFIED.,.F.,
 .F.,.F.)
B_SPLINE_SURFACE_WITH_KNOTS((4,4),(3,3),(2.71050543121376E-20,0.00039739446544831),
(0.,1.),.UNSPECIFIED.)
GEOMETRIC_REPRESENTATION_ITEM()
RATIONAL_B_SPLINE_SURFACE(((1.,0.705498956110749,1.),(1.,0.705821764811765,
1.),(1.,0.706461952521142,1.),(1.,0.707106781186548,1.)))
REPRESENTATION_ITEM('')
SURFACE()
);
#3586=(
BOUNDED_SURFACE()
B_SPLINE_SURFACE(3,2,((#247039,#247040,#247041),(#247042,#247043,#247044),
(#247045,#247046,#247047),(#247048,#247049,#247050)),.UNSPECIFIED.,.F.,
 .F.,.F.)
B_SPLINE_SURFACE_WITH_KNOTS((4,4),(3,3),(0.,0.000397394410828733),(0.,1.),
 .UNSPECIFIED.)
GEOMETRIC_REPRESENTATION_ITEM()
RATIONAL_B_SPLINE_SURFACE(((1.,0.708689770883331,1.),(1.,0.70837644003449,
1.),(1.,0.707750498698411,1.),(1.,0.707106781186548,1.)))
REPRESENTATION_ITEM('')
SURFACE()
);
#3587=(
BOUNDED_SURFACE()
B_SPLINE_SURFACE(3,2,((#247056,#247057,#247058),(#247059,#247060,#247061),
(#247062,#247063,#247064),(#247065,#247066,#247067)),.UNSPECIFIED.,.F.,
 .F.,.F.)
B_SPLINE_SURFACE_WITH_KNOTS((4,4),(3,3),(0.,0.000511815090126173),(0.,1.00105592270359),
 .UNSPECIFIED.)
GEOMETRIC_REPRESENTATION_ITEM()
RATIONAL_B_SPLINE_SURFACE(((1.,0.705266242717076,1.00062243213166),(1.,
0.705584085908736,1.00062176089597),(1.,0.70618208945009,1.00062049800494),
(1.,0.706797508587075,1.00061919833486)))
REPRESENTATION_ITEM('')
SURFACE()
);
#3588=(
BOUNDED_SURFACE()
B_SPLINE_SURFACE(3,2,((#247069,#247070,#247071),(#247072,#247073,#247074),
(#247075,#247076,#247077),(#247078,#247079,#247080)),.UNSPECIFIED.,.F.,
 .F.,.F.)
B_SPLINE_SURFACE_WITH_KNOTS((4,4),(3,3),(-7.07441917546792E-18,0.00039739442808662),
(0.,1.),.UNSPECIFIED.)
GEOMETRIC_REPRESENTATION_ITEM()
RATIONAL_B_SPLINE_SURFACE(((1.,0.707106781186548,1.),(1.,0.706459846759096,
1.),(1.,0.705820510737264,1.),(1.,0.705498956110752,1.)))
REPRESENTATION_ITEM('')
SURFACE()
);
#3589=(
BOUNDED_SURFACE()
B_SPLINE_SURFACE(3,2,((#247086,#247087,#247088),(#247089,#247090,#247091),
(#247092,#247093,#247094),(#247095,#247096,#247097),(#247098,#247099,#247100),
(#247101,#247102,#247103)),.UNSPECIFIED.,.F.,.F.,.F.)
B_SPLINE_SURFACE_WITH_KNOTS((4,2,4),(3,3),(-9.48676900924816E-20,0.000257953807872841,
0.000515907615745682),(0.,1.),.UNSPECIFIED.)
GEOMETRIC_REPRESENTATION_ITEM()
RATIONAL_B_SPLINE_SURFACE(((1.,0.874619707139395,1.),(1.,0.874834349678826,
1.),(1.,0.854686104158014,1.),(1.,0.792476597914929,1.),(1.,0.750887854595294,
1.),(1.,0.70558583803145,1.)))
REPRESENTATION_ITEM('')
SURFACE()
);
#3590=(
BOUNDED_SURFACE()
B_SPLINE_SURFACE(3,2,((#247106,#247107,#247108),(#247109,#247110,#247111),
(#247112,#247113,#247114),(#247115,#247116,#247117)),.UNSPECIFIED.,.F.,
 .F.,.F.)
B_SPLINE_SURFACE_WITH_KNOTS((4,4),(3,3),(0.,0.000511815437699145),(0.,1.00105881331498),
 .UNSPECIFIED.)
GEOMETRIC_REPRESENTATION_ITEM()
RATIONAL_B_SPLINE_SURFACE(((1.,0.706796661946602,1.00062089519665),(1.,
0.707430821225483,1.00061955228408),(1.,0.708058545830975,1.00061822299773),
(1.,0.708394505252982,1.00061751156112)))
REPRESENTATION_ITEM('')
SURFACE()
);
#3591=(
BOUNDED_SURFACE()
B_SPLINE_SURFACE(3,2,((#247119,#247120,#247121),(#247122,#247123,#247124),
(#247125,#247126,#247127),(#247128,#247129,#247130),(#247131,#247132,#247133),
(#247134,#247135,#247136)),.UNSPECIFIED.,.F.,.F.,.F.)
B_SPLINE_SURFACE_WITH_KNOTS((4,2,4),(3,3),(1.62630325872826E-19,0.00025691531753126,
0.00051383063506252),(0.,1.),.UNSPECIFIED.)
GEOMETRIC_REPRESENTATION_ITEM()
RATIONAL_B_SPLINE_SURFACE(((1.,0.705585838031442,1.),(1.,0.750902433542864,
1.),(1.,0.792329530082364,1.),(1.,0.854288401594348,1.),(1.,0.874998031125022,
1.),(1.,0.874619707139395,1.)))
REPRESENTATION_ITEM('')
SURFACE()
);
#3592=(
BOUNDED_SURFACE()
B_SPLINE_SURFACE(3,2,((#247142,#247143,#247144),(#247145,#247146,#247147),
(#247148,#247149,#247150),(#247151,#247152,#247153),(#247154,#247155,#247156),
(#247157,#247158,#247159)),.UNSPECIFIED.,.F.,.F.,.F.)
B_SPLINE_SURFACE_WITH_KNOTS((4,2,4),(3,3),(-1.32814766129474E-17,0.000256592814262149,
0.000513185628524311),(0.,1.),.UNSPECIFIED.)
GEOMETRIC_REPRESENTATION_ITEM()
RATIONAL_B_SPLINE_SURFACE(((1.,0.708712527163647,1.),(1.,0.75378090261363,
1.),(1.,0.794538995769148,1.),(1.,0.855070770331167,1.),(1.,0.87501842744528,
1.),(1.,0.874619707139394,1.)))
REPRESENTATION_ITEM('')
SURFACE()
);
#3593=(
BOUNDED_SURFACE()
B_SPLINE_SURFACE(3,2,((#247160,#247161,#247162),(#247163,#247164,#247165),
(#247166,#247167,#247168),(#247169,#247170,#247171)),.UNSPECIFIED.,.F.,
 .F.,.F.)
B_SPLINE_SURFACE_WITH_KNOTS((4,4),(3,3),(2.71050543121376E-20,0.000511815072430403),
(0.,1.0010559836588),.UNSPECIFIED.)
GEOMETRIC_REPRESENTATION_ITEM()
RATIONAL_B_SPLINE_SURFACE(((1.,0.706797490733709,1.00061923411701),(1.,
0.706182062146628,1.00062053388207),(1.,0.70558406276899,1.00062179683721),
(1.,0.705266224770469,1.00062246810067)))
REPRESENTATION_ITEM('')
SURFACE()
);
#3594=(
BOUNDED_SURFACE()
B_SPLINE_SURFACE(3,2,((#247175,#247176,#247177),(#247178,#247179,#247180),
(#247181,#247182,#247183),(#247184,#247185,#247186),(#247187,#247188,#247189),
(#247190,#247191,#247192)),.UNSPECIFIED.,.F.,.F.,.F.)
B_SPLINE_SURFACE_WITH_KNOTS((4,2,4),(3,3),(8.13151629364128E-20,0.000257652232350873,
0.000515304464701745),(0.,1.),.UNSPECIFIED.)
GEOMETRIC_REPRESENTATION_ITEM()
RATIONAL_B_SPLINE_SURFACE(((1.,0.8746197071394,1.),(1.,0.874861180430503,
1.),(1.,0.855455725921145,1.),(1.,0.79469935895498,1.),(1.,0.753768977788861,
1.),(1.,0.708712527163669,1.)))
REPRESENTATION_ITEM('')
SURFACE()
);
#3595=(
BOUNDED_SURFACE()
B_SPLINE_SURFACE(3,2,((#247198,#247199,#247200),(#247201,#247202,#247203),
(#247204,#247205,#247206),(#247207,#247208,#247209)),.UNSPECIFIED.,.F.,
 .F.,.F.)
B_SPLINE_SURFACE_WITH_KNOTS((4,4),(3,3),(0.,0.00039739437365191),(0.,1.),
 .UNSPECIFIED.)
GEOMETRIC_REPRESENTATION_ITEM()
RATIONAL_B_SPLINE_SURFACE(((1.,0.707106781186548,1.),(1.,0.707752587915901,
1.),(1.,0.708377654540677,1.),(1.,0.708689770883331,1.)))
REPRESENTATION_ITEM('')
SURFACE()
);
#3596=(
BOUNDED_SURFACE()
B_SPLINE_SURFACE(3,2,((#247211,#247212,#247213),(#247214,#247215,#247216),
(#247217,#247218,#247219),(#247220,#247221,#247222)),.UNSPECIFIED.,.F.,
 .F.,.F.)
B_SPLINE_SURFACE_WITH_KNOTS((4,4),(3,3),(-5.61074624261249E-18,0.000511815456479785),
(0.,1.00105873159895),.UNSPECIFIED.)
GEOMETRIC_REPRESENTATION_ITEM()
RATIONAL_B_SPLINE_SURFACE(((1.,0.70839452905662,1.00061746385303),(1.,0.708058564167168,
1.00061817524632),(1.,0.707430835372348,1.00061950443894),(1.,0.706796685880671,
1.00062084722715)))
REPRESENTATION_ITEM('')
SURFACE()
);
#3597=(
BOUNDED_SURFACE()
B_SPLINE_SURFACE(3,2,((#247228,#247229,#247230),(#247231,#247232,#247233),
(#247234,#247235,#247236),(#247237,#247238,#247239)),.UNSPECIFIED.,.F.,
 .F.,.F.)
B_SPLINE_SURFACE_WITH_KNOTS((4,4),(3,3),(0.,0.000397394465448314),(0.,1.),
 .UNSPECIFIED.)
GEOMETRIC_REPRESENTATION_ITEM()
RATIONAL_B_SPLINE_SURFACE(((1.,0.705498956110752,1.),(1.,0.705821764811787,
1.),(1.,0.706461952521144,1.),(1.,0.707106781186548,1.)))
REPRESENTATION_ITEM('')
SURFACE()
);
#3598=(
BOUNDED_SURFACE()
B_SPLINE_SURFACE(3,2,((#247245,#247246,#247247),(#247248,#247249,#247250),
(#247251,#247252,#247253),(#247254,#247255,#247256)),.UNSPECIFIED.,.F.,
 .F.,.F.)
B_SPLINE_SURFACE_WITH_KNOTS((4,4),(3,3),(2.71050543121376E-20,0.000397394410828732),
(0.,1.),.UNSPECIFIED.)
GEOMETRIC_REPRESENTATION_ITEM()
RATIONAL_B_SPLINE_SURFACE(((1.,0.708689770883327,1.),(1.,0.708376440034475,
1.),(1.,0.707750498698411,1.),(1.,0.707106781186548,1.)))
REPRESENTATION_ITEM('')
SURFACE()
);
#3599=(
BOUNDED_SURFACE()
B_SPLINE_SURFACE(3,2,((#247262,#247263,#247264),(#247265,#247266,#247267),
(#247268,#247269,#247270),(#247271,#247272,#247273)),.UNSPECIFIED.,.F.,
 .F.,.F.)
B_SPLINE_SURFACE_WITH_KNOTS((4,4),(3,3),(-2.71050543121376E-20,0.000511815090126174),
(0.,1.00105592270086),.UNSPECIFIED.)
GEOMETRIC_REPRESENTATION_ITEM()
RATIONAL_B_SPLINE_SURFACE(((1.,0.705266242717886,1.00062243213005),(1.,
0.705584085909542,1.00062176089437),(1.,0.706182089450896,1.00062049800334),
(1.,0.706797508587876,1.00061919833326)))
REPRESENTATION_ITEM('')
SURFACE()
);
#3600=(
BOUNDED_SURFACE()
B_SPLINE_SURFACE(3,2,((#247275,#247276,#247277),(#247278,#247279,#247280),
(#247281,#247282,#247283),(#247284,#247285,#247286)),.UNSPECIFIED.,.F.,
 .F.,.F.)
B_SPLINE_SURFACE_WITH_KNOTS((4,4),(3,3),(-7.02020906684364E-18,0.000397394428086623),
(0.,1.),.UNSPECIFIED.)
GEOMETRIC_REPRESENTATION_ITEM()
RATIONAL_B_SPLINE_SURFACE(((1.,0.707106781186548,1.),(1.,0.706459846759084,
1.),(1.,0.705820510737286,1.),(1.,0.705498956110757,1.)))
REPRESENTATION_ITEM('')
SURFACE()
);
#3601=(
BOUNDED_SURFACE()
B_SPLINE_SURFACE(3,2,((#247292,#247293,#247294),(#247295,#247296,#247297),
(#247298,#247299,#247300),(#247301,#247302,#247303),(#247304,#247305,#247306),
(#247307,#247308,#247309)),.UNSPECIFIED.,.F.,.F.,.F.)
B_SPLINE_SURFACE_WITH_KNOTS((4,2,4),(3,3),(-8.53809210832335E-19,0.000257953807872841,
0.000515907615745684),(0.,1.),.UNSPECIFIED.)
GEOMETRIC_REPRESENTATION_ITEM()
RATIONAL_B_SPLINE_SURFACE(((1.,0.87461970713939,1.),(1.,0.874834349679068,
1.),(1.,0.854686104157704,1.),(1.,0.792476597915263,1.),(1.,0.750887854595055,
1.),(1.,0.705585838031452,1.)))
REPRESENTATION_ITEM('')
SURFACE()
);
#3602=(
BOUNDED_SURFACE()
B_SPLINE_SURFACE(3,2,((#247315,#247316,#247317),(#247318,#247319,#247320),
(#247321,#247322,#247323),(#247324,#247325,#247326)),.UNSPECIFIED.,.F.,
 .F.,.F.)
B_SPLINE_SURFACE_WITH_KNOTS((4,4),(3,3),(-1.0842021724855E-19,0.000511815437699153),
(0.,1.00105881331538),.UNSPECIFIED.)
GEOMETRIC_REPRESENTATION_ITEM()
RATIONAL_B_SPLINE_SURFACE(((1.,0.706796661946481,1.00062089519689),(1.,
0.707430821225356,1.00061955228431),(1.,0.708058545830853,1.00061822299797),
(1.,0.708394505252858,1.00061751156135)))
REPRESENTATION_ITEM('')
SURFACE()
);
#3603=(
BOUNDED_SURFACE()
B_SPLINE_SURFACE(3,2,((#247328,#247329,#247330),(#247331,#247332,#247333),
(#247334,#247335,#247336),(#247337,#247338,#247339),(#247340,#247341,#247342),
(#247343,#247344,#247345)),.UNSPECIFIED.,.F.,.F.,.F.)
B_SPLINE_SURFACE_WITH_KNOTS((4,2,4),(3,3),(1.0842021724855E-19,0.000256915317531263,
0.000513830635062526),(0.,1.),.UNSPECIFIED.)
GEOMETRIC_REPRESENTATION_ITEM()
RATIONAL_B_SPLINE_SURFACE(((1.,0.70558583803143,1.),(1.,0.750902433542735,
1.),(1.,0.792329530082518,1.),(1.,0.854288401594187,1.),(1.,0.874998031125162,
1.),(1.,0.874619707139389,1.)))
REPRESENTATION_ITEM('')
SURFACE()
);
#3604=(
BOUNDED_SURFACE()
B_SPLINE_SURFACE(3,2,((#247351,#247352,#247353),(#247354,#247355,#247356),
(#247357,#247358,#247359),(#247360,#247361,#247362),(#247363,#247364,#247365),
(#247366,#247367,#247368)),.UNSPECIFIED.,.F.,.F.,.F.)
B_SPLINE_SURFACE_WITH_KNOTS((4,2,4),(3,3),(-1.04625509644851E-17,0.00025659281426215,
0.000513185628524311),(0.,1.),.UNSPECIFIED.)
GEOMETRIC_REPRESENTATION_ITEM()
RATIONAL_B_SPLINE_SURFACE(((1.,0.708712527163659,1.),(1.,0.753780902613745,
1.),(1.,0.794538995768978,1.),(1.,0.855070770331331,1.),(1.,0.875018427445157,
1.),(1.,0.874619707139395,1.)))
REPRESENTATION_ITEM('')
SURFACE()
);
#3605=(
BOUNDED_SURFACE()
B_SPLINE_SURFACE(3,2,((#247370,#247371,#247372),(#247373,#247374,#247375),
(#247376,#247377,#247378),(#247379,#247380,#247381)),.UNSPECIFIED.,.F.,
 .F.,.F.)
B_SPLINE_SURFACE_WITH_KNOTS((4,4),(3,3),(-7.61652026171067E-18,0.00051181507243039),
(0.,1.00105598365716),.UNSPECIFIED.)
GEOMETRIC_REPRESENTATION_ITEM()
RATIONAL_B_SPLINE_SURFACE(((1.,0.706797490734189,1.00061923411605),(1.,
0.7061820621471,1.00062053388111),(1.,0.705584062769466,1.00062179683625),
(1.,0.705266224770944,1.00062246809971)))
REPRESENTATION_ITEM('')
SURFACE()
);
#3606=(
BOUNDED_SURFACE()
B_SPLINE_SURFACE(3,2,((#247387,#247388,#247389),(#247390,#247391,#247392),
(#247393,#247394,#247395),(#247396,#247397,#247398),(#247399,#247400,#247401),
(#247402,#247403,#247404)),.UNSPECIFIED.,.F.,.F.,.F.)
B_SPLINE_SURFACE_WITH_KNOTS((4,2,4),(3,3),(-2.62919026827735E-18,0.000257652232350876,
0.000515304464701754),(0.,1.),.UNSPECIFIED.)
GEOMETRIC_REPRESENTATION_ITEM()
RATIONAL_B_SPLINE_SURFACE(((1.,0.874619707139396,1.),(1.,0.874861180430993,
1.),(1.,0.855455725920489,1.),(1.,0.794699358955656,1.),(1.,0.753768977788361,
1.),(1.,0.708712527163659,1.)))
REPRESENTATION_ITEM('')
SURFACE()
);
#3607=(
BOUNDED_SURFACE()
B_SPLINE_SURFACE(3,2,((#247410,#247411,#247412),(#247413,#247414,#247415),
(#247416,#247417,#247418),(#247419,#247420,#247421)),.UNSPECIFIED.,.F.,
 .F.,.F.)
B_SPLINE_SURFACE_WITH_KNOTS((4,4),(3,3),(-7.18283939271647E-18,0.000397394373651905),
(0.,1.),.UNSPECIFIED.)
GEOMETRIC_REPRESENTATION_ITEM()
RATIONAL_B_SPLINE_SURFACE(((1.,0.707106781186548,1.),(1.,0.707752587915914,
1.),(1.,0.70837765454066,1.),(1.,0.708689770883359,1.)))
REPRESENTATION_ITEM('')
SURFACE()
);
#3608=(
BOUNDED_SURFACE()
B_SPLINE_SURFACE(3,2,((#247423,#247424,#247425),(#247426,#247427,#247428),
(#247429,#247430,#247431),(#247432,#247433,#247434)),.UNSPECIFIED.,.F.,
 .F.,.F.)
B_SPLINE_SURFACE_WITH_KNOTS((4,4),(3,3),(5.42101086242752E-20,0.000511815456479787),
(0.,1.00105873159955),.UNSPECIFIED.)
GEOMETRIC_REPRESENTATION_ITEM()
RATIONAL_B_SPLINE_SURFACE(((1.,0.708394529056452,1.00061746385338),(1.,
0.708058564166979,1.00061817524667),(1.,0.707430835372198,1.00061950443929),
(1.,0.706796685880492,1.0006208472275)))
REPRESENTATION_ITEM('')
SURFACE()
);
#3609=(
BOUNDED_SURFACE()
B_SPLINE_SURFACE(3,2,((#247440,#247441,#247442),(#247443,#247444,#247445),
(#247446,#247447,#247448),(#247449,#247450,#247451)),.UNSPECIFIED.,.F.,
 .F.,.F.)
B_SPLINE_SURFACE_WITH_KNOTS((4,4),(3,3),(-2.71050543121376E-20,0.00039739446544831),
(0.,1.),.UNSPECIFIED.)
GEOMETRIC_REPRESENTATION_ITEM()
RATIONAL_B_SPLINE_SURFACE(((1.,0.705498956110745,1.),(1.,0.705821764811779,
1.),(1.,0.706461952521128,1.),(1.,0.70710678118655,1.)))
REPRESENTATION_ITEM('')
SURFACE()
);
#3610=(
BOUNDED_SURFACE()
B_SPLINE_SURFACE(3,2,((#247457,#247458,#247459),(#247460,#247461,#247462),
(#247463,#247464,#247465),(#247466,#247467,#247468)),.UNSPECIFIED.,.F.,
 .F.,.F.)
B_SPLINE_SURFACE_WITH_KNOTS((4,4),(3,3),(0.,0.00039739441082874),(0.,1.),
 .UNSPECIFIED.)
GEOMETRIC_REPRESENTATION_ITEM()
RATIONAL_B_SPLINE_SURFACE(((1.,0.708689770883333,1.),(1.,0.708376440034488,
1.),(1.,0.707750498698412,1.),(1.,0.70710678118655,1.)))
REPRESENTATION_ITEM('')
SURFACE()
);
#3611=(
BOUNDED_SURFACE()
B_SPLINE_SURFACE(3,2,((#247474,#247475,#247476),(#247477,#247478,#247479),
(#247480,#247481,#247482),(#247483,#247484,#247485)),.UNSPECIFIED.,.F.,
 .F.,.F.)
B_SPLINE_SURFACE_WITH_KNOTS((4,4),(3,3),(-1.35525271560688E-19,0.000511815090126177),
(0.,1.00105592270234),.UNSPECIFIED.)
GEOMETRIC_REPRESENTATION_ITEM()
RATIONAL_B_SPLINE_SURFACE(((1.,0.70526624271744,1.00062243213092),(1.,0.705584085909104,
1.00062176089524),(1.,0.706182089450463,1.0006204980042),(1.,0.70679750858744,
1.00061919833413)))
REPRESENTATION_ITEM('')
SURFACE()
);
#3612=(
BOUNDED_SURFACE()
B_SPLINE_SURFACE(3,2,((#247487,#247488,#247489),(#247490,#247491,#247492),
(#247493,#247494,#247495),(#247496,#247497,#247498)),.UNSPECIFIED.,.F.,
 .F.,.F.)
B_SPLINE_SURFACE_WITH_KNOTS((4,4),(3,3),(0.,0.000397394428086621),(0.,1.),
 .UNSPECIFIED.)
GEOMETRIC_REPRESENTATION_ITEM()
RATIONAL_B_SPLINE_SURFACE(((1.,0.707106781186545,1.),(1.,0.706459846759102,
1.),(1.,0.705820510737278,1.),(1.,0.705498956110747,1.)))
REPRESENTATION_ITEM('')
SURFACE()
);
#3613=(
BOUNDED_SURFACE()
B_SPLINE_SURFACE(3,2,((#247504,#247505,#247506),(#247507,#247508,#247509),
(#247510,#247511,#247512),(#247513,#247514,#247515),(#247516,#247517,#247518),
(#247519,#247520,#247521)),.UNSPECIFIED.,.F.,.F.,.F.)
B_SPLINE_SURFACE_WITH_KNOTS((4,2,4),(3,3),(0.,0.000257953807872835,0.000515907615745671),
(0.,1.),.UNSPECIFIED.)
GEOMETRIC_REPRESENTATION_ITEM()
RATIONAL_B_SPLINE_SURFACE(((1.,0.874619707139395,1.),(1.,0.874834349678973,
1.),(1.,0.854686104157817,1.),(1.,0.792476597915156,1.),(1.,0.750887854595112,
1.),(1.,0.705585838031439,1.)))
REPRESENTATION_ITEM('')
SURFACE()
);
#3614=(
BOUNDED_SURFACE()
B_SPLINE_SURFACE(3,2,((#247527,#247528,#247529),(#247530,#247531,#247532),
(#247533,#247534,#247535),(#247536,#247537,#247538)),.UNSPECIFIED.,.F.,
 .F.,.F.)
B_SPLINE_SURFACE_WITH_KNOTS((4,4),(3,3),(0.,0.000511815437699155),(0.,1.0010588133155),
 .UNSPECIFIED.)
GEOMETRIC_REPRESENTATION_ITEM()
RATIONAL_B_SPLINE_SURFACE(((1.,0.706796661946457,1.00062089519696),(1.,
0.707430821225312,1.00061955228438),(1.,0.708058545830853,1.00061822299804),
(1.,0.708394505252833,1.00061751156142)))
REPRESENTATION_ITEM('')
SURFACE()
);
#3615=(
BOUNDED_SURFACE()
B_SPLINE_SURFACE(3,2,((#247540,#247541,#247542),(#247543,#247544,#247545),
(#247546,#247547,#247548),(#247549,#247550,#247551),(#247552,#247553,#247554),
(#247555,#247556,#247557)),.UNSPECIFIED.,.F.,.F.,.F.)
B_SPLINE_SURFACE_WITH_KNOTS((4,2,4),(3,3),(0.,0.00025691531753126,0.00051383063506252),
(0.,1.),.UNSPECIFIED.)
GEOMETRIC_REPRESENTATION_ITEM()
RATIONAL_B_SPLINE_SURFACE(((1.,0.705585838031444,1.),(1.,0.750902433542275,
1.),(1.,0.792329530083157,1.),(1.,0.854288401593573,1.),(1.,0.87499803112561,
1.),(1.,0.874619707139394,1.)))
REPRESENTATION_ITEM('')
SURFACE()
);
#3616=(
BOUNDED_SURFACE()
B_SPLINE_SURFACE(3,2,((#247563,#247564,#247565),(#247566,#247567,#247568),
(#247569,#247570,#247571),(#247572,#247573,#247574),(#247575,#247576,#247577),
(#247578,#247579,#247580)),.UNSPECIFIED.,.F.,.F.,.F.)
B_SPLINE_SURFACE_WITH_KNOTS((4,2,4),(3,3),(0.,0.000256592814262163,0.000513185628524326),
(0.,1.),.UNSPECIFIED.)
GEOMETRIC_REPRESENTATION_ITEM()
RATIONAL_B_SPLINE_SURFACE(((1.,0.708712527163656,1.),(1.,0.7537809026137,
1.),(1.,0.794538995769058,1.),(1.,0.855070770331249,1.),(1.,0.875018427445215,
1.),(1.,0.874619707139403,1.)))
REPRESENTATION_ITEM('')
SURFACE()
);
#3617=(
BOUNDED_SURFACE()
B_SPLINE_SURFACE(3,2,((#247582,#247583,#247584),(#247585,#247586,#247587),
(#247588,#247589,#247590),(#247591,#247592,#247593)),.UNSPECIFIED.,.F.,
 .F.,.F.)
B_SPLINE_SURFACE_WITH_KNOTS((4,4),(3,3),(0.,0.0005118150724304),(0.,1.00105598365535),
 .UNSPECIFIED.)
GEOMETRIC_REPRESENTATION_ITEM()
RATIONAL_B_SPLINE_SURFACE(((1.,0.706797490734715,1.00061923411498),(1.,
0.706182062147634,1.00062053388004),(1.,0.705584062770011,1.00062179683518),
(1.,0.705266224771485,1.00062246809864)))
REPRESENTATION_ITEM('')
SURFACE()
);
#3618=(
BOUNDED_SURFACE()
B_SPLINE_SURFACE(3,2,((#247599,#247600,#247601),(#247602,#247603,#247604),
(#247605,#247606,#247607),(#247608,#247609,#247610),(#247611,#247612,#247613),
(#247614,#247615,#247616)),.UNSPECIFIED.,.F.,.F.,.F.)
B_SPLINE_SURFACE_WITH_KNOTS((4,2,4),(3,3),(-3.46944695195361E-18,0.000257652232350873,
0.00051530446470175),(0.,1.),.UNSPECIFIED.)
GEOMETRIC_REPRESENTATION_ITEM()
RATIONAL_B_SPLINE_SURFACE(((1.,0.874619707139393,1.),(1.,0.874861180430414,
1.),(1.,0.855455725921246,1.),(1.,0.794699358954878,1.),(1.,0.753768977788917,
1.),(1.,0.708712527163685,1.)))
REPRESENTATION_ITEM('')
SURFACE()
);
#3619=(
BOUNDED_SURFACE()
B_SPLINE_SURFACE(3,2,((#247622,#247623,#247624),(#247625,#247626,#247627),
(#247628,#247629,#247630),(#247631,#247632,#247633)),.UNSPECIFIED.,.F.,
 .F.,.F.)
B_SPLINE_SURFACE_WITH_KNOTS((4,4),(3,3),(0.,0.000397394373651924),(0.,1.),
 .UNSPECIFIED.)
GEOMETRIC_REPRESENTATION_ITEM()
RATIONAL_B_SPLINE_SURFACE(((1.,0.70710678118655,1.),(1.,0.707752587915898,
1.),(1.,0.708377654540676,1.),(1.,0.708689770883331,1.)))
REPRESENTATION_ITEM('')
SURFACE()
);
#3620=(
BOUNDED_SURFACE()
B_SPLINE_SURFACE(3,2,((#247635,#247636,#247637),(#247638,#247639,#247640),
(#247641,#247642,#247643),(#247644,#247645,#247646)),.UNSPECIFIED.,.F.,
 .F.,.F.)
B_SPLINE_SURFACE_WITH_KNOTS((4,4),(3,3),(-3.06287113727155E-18,0.000511815456479783),
(0.,1.00105873159907),.UNSPECIFIED.)
GEOMETRIC_REPRESENTATION_ITEM()
RATIONAL_B_SPLINE_SURFACE(((1.,0.708394529056585,1.0006174638531),(1.,0.708058564167109,
1.00061817524639),(1.,0.707430835372329,1.00061950443901),(1.,0.706796685880633,
1.00062084722722)))
REPRESENTATION_ITEM('')
SURFACE()
);
#3621=(
BOUNDED_SURFACE()
B_SPLINE_SURFACE(3,2,((#247652,#247653,#247654),(#247655,#247656,#247657),
(#247658,#247659,#247660),(#247661,#247662,#247663)),.UNSPECIFIED.,.F.,
 .F.,.F.)
B_SPLINE_SURFACE_WITH_KNOTS((4,4),(3,3),(0.,0.000397394465448322),(0.,1.),
 .UNSPECIFIED.)
GEOMETRIC_REPRESENTATION_ITEM()
RATIONAL_B_SPLINE_SURFACE(((1.,0.705498956110758,1.),(1.,0.705821764811796,
1.),(1.,0.706461952521131,1.),(1.,0.707106781186554,1.)))
REPRESENTATION_ITEM('')
SURFACE()
);
#3622=(
BOUNDED_SURFACE()
B_SPLINE_SURFACE(3,2,((#247669,#247670,#247671),(#247672,#247673,#247674),
(#247675,#247676,#247677),(#247678,#247679,#247680)),.UNSPECIFIED.,.F.,
 .F.,.F.)
B_SPLINE_SURFACE_WITH_KNOTS((4,4),(3,3),(3.79470760369927E-19,0.000397394410828729),
(0.,1.),.UNSPECIFIED.)
GEOMETRIC_REPRESENTATION_ITEM()
RATIONAL_B_SPLINE_SURFACE(((1.,0.708689770883329,1.),(1.,0.708376440034479,
1.),(1.,0.707750498698412,1.),(1.,0.70710678118655,1.)))
REPRESENTATION_ITEM('')
SURFACE()
);
#3623=(
BOUNDED_SURFACE()
B_SPLINE_SURFACE(3,2,((#247686,#247687,#247688),(#247689,#247690,#247691),
(#247692,#247693,#247694),(#247695,#247696,#247697)),.UNSPECIFIED.,.F.,
 .F.,.F.)
B_SPLINE_SURFACE_WITH_KNOTS((4,4),(3,3),(0.,0.000511815090126172),(0.,1.00105592270453),
 .UNSPECIFIED.)
GEOMETRIC_REPRESENTATION_ITEM()
RATIONAL_B_SPLINE_SURFACE(((1.,0.705266242716804,1.00062243213221),(1.,
0.705584085908435,1.00062176089653),(1.,0.706182089449835,1.0006204980055),
(1.,0.706797508586802,1.00061919833542)))
REPRESENTATION_ITEM('')
SURFACE()
);
#3624=(
BOUNDED_SURFACE()
B_SPLINE_SURFACE(3,2,((#247699,#247700,#247701),(#247702,#247703,#247704),
(#247705,#247706,#247707),(#247708,#247709,#247710)),.UNSPECIFIED.,.F.,
 .F.,.F.)
B_SPLINE_SURFACE_WITH_KNOTS((4,4),(3,3),(-7.80625564189563E-18,0.000397394428086628),
(0.,1.),.UNSPECIFIED.)
GEOMETRIC_REPRESENTATION_ITEM()
RATIONAL_B_SPLINE_SURFACE(((1.,0.70710678118655,1.),(1.,0.70645984675907,
1.),(1.,0.705820510737293,1.),(1.,0.705498956110754,1.)))
REPRESENTATION_ITEM('')
SURFACE()
);
#3625=(
BOUNDED_SURFACE()
B_SPLINE_SURFACE(3,2,((#247716,#247717,#247718),(#247719,#247720,#247721),
(#247722,#247723,#247724),(#247725,#247726,#247727),(#247728,#247729,#247730),
(#247731,#247732,#247733)),.UNSPECIFIED.,.F.,.F.,.F.)
B_SPLINE_SURFACE_WITH_KNOTS((4,2,4),(3,3),(0.,0.00025795380787285,0.000515907615745699),
(0.,1.),.UNSPECIFIED.)
GEOMETRIC_REPRESENTATION_ITEM()
RATIONAL_B_SPLINE_SURFACE(((1.,0.874619707139402,1.),(1.,0.874834349679344,
1.),(1.,0.854686104157338,1.),(1.,0.792476597915597,1.),(1.,0.750887854594773,
1.),(1.,0.705585838031445,1.)))
REPRESENTATION_ITEM('')
SURFACE()
);
#3626=(
BOUNDED_SURFACE()
B_SPLINE_SURFACE(3,2,((#247739,#247740,#247741),(#247742,#247743,#247744),
(#247745,#247746,#247747),(#247748,#247749,#247750)),.UNSPECIFIED.,.F.,
 .F.,.F.)
B_SPLINE_SURFACE_WITH_KNOTS((4,4),(3,3),(-8.13151629364128E-20,0.000511815437699148),
(0.,1.00105881331685),.UNSPECIFIED.)
GEOMETRIC_REPRESENTATION_ITEM()
RATIONAL_B_SPLINE_SURFACE(((1.,0.706796661946055,1.00062089519775),(1.,
0.707430821224927,1.00061955228517),(1.,0.708058545830431,1.00061822299883),
(1.,0.708394505252429,1.00061751156221)))
REPRESENTATION_ITEM('')
SURFACE()
);
#3627=(
BOUNDED_SURFACE()
B_SPLINE_SURFACE(3,2,((#247752,#247753,#247754),(#247755,#247756,#247757),
(#247758,#247759,#247760),(#247761,#247762,#247763),(#247764,#247765,#247766),
(#247767,#247768,#247769)),.UNSPECIFIED.,.F.,.F.,.F.)
B_SPLINE_SURFACE_WITH_KNOTS((4,2,4),(3,3),(5.42101086242752E-20,0.00025691531753127,
0.000513830635062541),(0.,1.),.UNSPECIFIED.)
GEOMETRIC_REPRESENTATION_ITEM()
RATIONAL_B_SPLINE_SURFACE(((1.,0.705585838031452,1.),(1.,0.750902433542135,
1.),(1.,0.792329530083361,1.),(1.,0.85428840159336,1.),(1.,0.874998031125796,
1.),(1.,0.874619707139413,1.)))
REPRESENTATION_ITEM('')
SURFACE()
);
#3628=(
BOUNDED_SURFACE()
B_SPLINE_SURFACE(3,2,((#247775,#247776,#247777),(#247778,#247779,#247780),
(#247781,#247782,#247783),(#247784,#247785,#247786),(#247787,#247788,#247789),
(#247790,#247791,#247792)),.UNSPECIFIED.,.F.,.F.,.F.)
B_SPLINE_SURFACE_WITH_KNOTS((4,2,4),(3,3),(-1.33085816672596E-17,0.000256592814262153,
0.000513185628524318),(0.,1.),.UNSPECIFIED.)
GEOMETRIC_REPRESENTATION_ITEM()
RATIONAL_B_SPLINE_SURFACE(((1.,0.708712527163657,1.),(1.,0.753780902613274,
1.),(1.,0.794538995769617,1.),(1.,0.855070770330683,1.),(1.,0.875018427445638,
1.),(1.,0.874619707139398,1.)))
REPRESENTATION_ITEM('')
SURFACE()
);
#3629=(
BOUNDED_SURFACE()
B_SPLINE_SURFACE(3,2,((#247794,#247795,#247796),(#247797,#247798,#247799),
(#247800,#247801,#247802),(#247803,#247804,#247805)),.UNSPECIFIED.,.F.,
 .F.,.F.)
B_SPLINE_SURFACE_WITH_KNOTS((4,4),(3,3),(0.,0.000511815072430392),(0.,1.00105598365709),
 .UNSPECIFIED.)
GEOMETRIC_REPRESENTATION_ITEM()
RATIONAL_B_SPLINE_SURFACE(((1.,0.706797490734206,1.000619234116),(1.,0.706182062147127,
1.00062053388107),(1.,0.705584062769492,1.0006217968362),(1.,0.705266224770968,
1.00062246809967)))
REPRESENTATION_ITEM('')
SURFACE()
);
#3630=(
BOUNDED_SURFACE()
B_SPLINE_SURFACE(3,2,((#247811,#247812,#247813),(#247814,#247815,#247816),
(#247817,#247818,#247819),(#247820,#247821,#247822),(#247823,#247824,#247825),
(#247826,#247827,#247828)),.UNSPECIFIED.,.F.,.F.,.F.)
B_SPLINE_SURFACE_WITH_KNOTS((4,2,4),(3,3),(0.,0.000257652232350887,0.000515304464701773),
(0.,1.),.UNSPECIFIED.)
GEOMETRIC_REPRESENTATION_ITEM()
RATIONAL_B_SPLINE_SURFACE(((1.,0.87461970713938,1.),(1.,0.874861180430769,
1.),(1.,0.855455725920777,1.),(1.,0.794699358955329,1.),(1.,0.753768977788596,
1.),(1.,0.708712527163624,1.)))
REPRESENTATION_ITEM('')
SURFACE()
);
#3631=(
BOUNDED_SURFACE()
B_SPLINE_SURFACE(3,2,((#247834,#247835,#247836),(#247837,#247838,#247839),
(#247840,#247841,#247842),(#247843,#247844,#247845)),.UNSPECIFIED.,.F.,
 .F.,.F.)
B_SPLINE_SURFACE_WITH_KNOTS((4,4),(3,3),(0.,0.000397394373651907),(0.,1.),
 .UNSPECIFIED.)
GEOMETRIC_REPRESENTATION_ITEM()
RATIONAL_B_SPLINE_SURFACE(((1.,0.707106781186545,1.),(1.,0.707752587915894,
1.),(1.,0.708377654540684,1.),(1.,0.708689770883333,1.)))
REPRESENTATION_ITEM('')
SURFACE()
);
#3632=(
BOUNDED_SURFACE()
B_SPLINE_SURFACE(3,2,((#247847,#247848,#247849),(#247850,#247851,#247852),
(#247853,#247854,#247855),(#247856,#247857,#247858)),.UNSPECIFIED.,.F.,
 .F.,.F.)
B_SPLINE_SURFACE_WITH_KNOTS((4,4),(3,3),(0.,0.000511815456479797),(0.,1.00105873160002),
 .UNSPECIFIED.)
GEOMETRIC_REPRESENTATION_ITEM()
RATIONAL_B_SPLINE_SURFACE(((1.,0.708394529056337,1.00061746385365),(1.,
0.708058564166813,1.00061817524694),(1.,0.707430835372066,1.00061950443957),
(1.,0.706796685880356,1.00062084722778)))
REPRESENTATION_ITEM('')
SURFACE()
);
#3633=(
BOUNDED_SURFACE()
B_SPLINE_SURFACE(3,2,((#247864,#247865,#247866),(#247867,#247868,#247869),
(#247870,#247871,#247872),(#247873,#247874,#247875)),.UNSPECIFIED.,.F.,
 .F.,.F.)
B_SPLINE_SURFACE_WITH_KNOTS((4,4),(3,3),(-3.52365706057789E-19,0.000397394465448304),
(0.,1.),.UNSPECIFIED.)
GEOMETRIC_REPRESENTATION_ITEM()
RATIONAL_B_SPLINE_SURFACE(((1.,0.705498956110757,1.),(1.,0.705821764811772,
1.),(1.,0.706461952521142,1.),(1.,0.707106781186548,1.)))
REPRESENTATION_ITEM('')
SURFACE()
);
#3634=(
BOUNDED_SURFACE()
B_SPLINE_SURFACE(3,2,((#247881,#247882,#247883),(#247884,#247885,#247886),
(#247887,#247888,#247889),(#247890,#247891,#247892)),.UNSPECIFIED.,.F.,
 .F.,.F.)
B_SPLINE_SURFACE_WITH_KNOTS((4,4),(3,3),(4.87890977618477E-19,0.000397394410828734),
(0.,1.),.UNSPECIFIED.)
GEOMETRIC_REPRESENTATION_ITEM()
RATIONAL_B_SPLINE_SURFACE(((1.,0.708689770883329,1.),(1.,0.708376440034481,
1.),(1.,0.707750498698425,1.),(1.,0.707106781186533,1.)))
REPRESENTATION_ITEM('')
SURFACE()
);
#3635=(
BOUNDED_SURFACE()
B_SPLINE_SURFACE(3,2,((#247898,#247899,#247900),(#247901,#247902,#247903),
(#247904,#247905,#247906),(#247907,#247908,#247909)),.UNSPECIFIED.,.F.,
 .F.,.F.)
B_SPLINE_SURFACE_WITH_KNOTS((4,4),(3,3),(3.19839640883224E-18,0.000511815090126191),
(0.,1.00105592270058),.UNSPECIFIED.)
GEOMETRIC_REPRESENTATION_ITEM()
RATIONAL_B_SPLINE_SURFACE(((1.,0.705266242717954,1.00062243212989),(1.,
0.705584085909609,1.0006217608942),(1.,0.706182089450989,1.00062049800317),
(1.,0.706797508587958,1.0006191983331)))
REPRESENTATION_ITEM('')
SURFACE()
);
#3636=(
BOUNDED_SURFACE()
B_SPLINE_SURFACE(3,2,((#247911,#247912,#247913),(#247914,#247915,#247916),
(#247917,#247918,#247919),(#247920,#247921,#247922)),.UNSPECIFIED.,.F.,
 .F.,.F.)
B_SPLINE_SURFACE_WITH_KNOTS((4,4),(3,3),(0.,0.00039739442808663),(0.,1.),
 .UNSPECIFIED.)
GEOMETRIC_REPRESENTATION_ITEM()
RATIONAL_B_SPLINE_SURFACE(((1.,0.70710678118655,1.),(1.,0.706459846759083,
1.),(1.,0.705820510737299,1.),(1.,0.705498956110753,1.)))
REPRESENTATION_ITEM('')
SURFACE()
);
#3637=(
BOUNDED_SURFACE()
B_SPLINE_SURFACE(3,2,((#247928,#247929,#247930),(#247931,#247932,#247933),
(#247934,#247935,#247936),(#247937,#247938,#247939),(#247940,#247941,#247942),
(#247943,#247944,#247945)),.UNSPECIFIED.,.F.,.F.,.F.)
B_SPLINE_SURFACE_WITH_KNOTS((4,2,4),(3,3),(0.,0.000257953807872844,0.000515907615745688),
(0.,1.),.UNSPECIFIED.)
GEOMETRIC_REPRESENTATION_ITEM()
RATIONAL_B_SPLINE_SURFACE(((1.,0.874619707139388,1.),(1.,0.874834349679326,
1.),(1.,0.854686104157358,1.),(1.,0.79247659791558,1.),(1.,0.750887854594821,
1.),(1.,0.705585838031413,1.)))
REPRESENTATION_ITEM('')
SURFACE()
);
#3638=(
BOUNDED_SURFACE()
B_SPLINE_SURFACE(3,2,((#247951,#247952,#247953),(#247954,#247955,#247956),
(#247957,#247958,#247959),(#247960,#247961,#247962)),.UNSPECIFIED.,.F.,
 .F.,.F.)
B_SPLINE_SURFACE_WITH_KNOTS((4,4),(3,3),(0.,0.000511815437699147),(0.,1.00105881331661),
 .UNSPECIFIED.)
GEOMETRIC_REPRESENTATION_ITEM()
RATIONAL_B_SPLINE_SURFACE(((1.,0.706796661946126,1.00062089519761),(1.,
0.707430821224989,1.00061955228503),(1.,0.708058545830522,1.00061822299869),
(1.,0.708394505252503,1.00061751156207)))
REPRESENTATION_ITEM('')
SURFACE()
);
#3639=(
BOUNDED_SURFACE()
B_SPLINE_SURFACE(3,2,((#247964,#247965,#247966),(#247967,#247968,#247969),
(#247970,#247971,#247972),(#247973,#247974,#247975),(#247976,#247977,#247978),
(#247979,#247980,#247981)),.UNSPECIFIED.,.F.,.F.,.F.)
B_SPLINE_SURFACE_WITH_KNOTS((4,2,4),(3,3),(-1.35525271560688E-19,0.000256915317531268,
0.000513830635062535),(0.,1.),.UNSPECIFIED.)
GEOMETRIC_REPRESENTATION_ITEM()
RATIONAL_B_SPLINE_SURFACE(((1.,0.705585838031459,1.),(1.,0.750902433542557,
1.),(1.,0.792329530082764,1.),(1.,0.854288401593981,1.),(1.,0.874998031125318,
1.),(1.,0.87461970713942,1.)))
REPRESENTATION_ITEM('')
SURFACE()
);
#3640=(
BOUNDED_SURFACE()
B_SPLINE_SURFACE(3,2,((#247987,#247988,#247989),(#247990,#247991,#247992),
(#247993,#247994,#247995),(#247996,#247997,#247998),(#247999,#248000,#248001),
(#248002,#248003,#248004)),.UNSPECIFIED.,.F.,.F.,.F.)
B_SPLINE_SURFACE_WITH_KNOTS((4,2,4),(3,3),(-1.05438661274215E-17,0.000256592814262151,
0.000513185628524312),(0.,1.),.UNSPECIFIED.)
GEOMETRIC_REPRESENTATION_ITEM()
RATIONAL_B_SPLINE_SURFACE(((1.,0.708712527163662,1.),(1.,0.753780902614111,
1.),(1.,0.79453899576847,1.),(1.,0.855070770331844,1.),(1.,0.875018427444773,
1.),(1.,0.874619707139394,1.)))
REPRESENTATION_ITEM('')
SURFACE()
);
#3641=(
BOUNDED_SURFACE()
B_SPLINE_SURFACE(3,2,((#248006,#248007,#248008),(#248009,#248010,#248011),
(#248012,#248013,#248014),(#248015,#248016,#248017)),.UNSPECIFIED.,.F.,
 .F.,.F.)
B_SPLINE_SURFACE_WITH_KNOTS((4,4),(3,3),(-5.42101086242752E-20,0.000511815072430393),
(0.,1.00105598365896),.UNSPECIFIED.)
GEOMETRIC_REPRESENTATION_ITEM()
RATIONAL_B_SPLINE_SURFACE(((1.,0.706797490733667,1.0006192341171),(1.,0.706182062146547,
1.00062053388216),(1.,0.705584062768983,1.0006217968373),(1.,0.70526622477041,
1.00062246810077)))
REPRESENTATION_ITEM('')
SURFACE()
);
#3642=(
BOUNDED_SURFACE()
B_SPLINE_SURFACE(3,2,((#248023,#248024,#248025),(#248026,#248027,#248028),
(#248029,#248030,#248031),(#248032,#248033,#248034),(#248035,#248036,#248037),
(#248038,#248039,#248040)),.UNSPECIFIED.,.F.,.F.,.F.)
B_SPLINE_SURFACE_WITH_KNOTS((4,2,4),(3,3),(-5.28548559086683E-19,0.000257652232350884,
0.000515304464701769),(0.,1.),.UNSPECIFIED.)
GEOMETRIC_REPRESENTATION_ITEM()
RATIONAL_B_SPLINE_SURFACE(((1.,0.87461970713938,1.),(1.,0.874861180430975,
1.),(1.,0.855455725920509,1.),(1.,0.794699358955589,1.),(1.,0.753768977788371,
1.),(1.,0.708712527163643,1.)))
REPRESENTATION_ITEM('')
SURFACE()
);
#3643=(
BOUNDED_SURFACE()
B_SPLINE_SURFACE(3,2,((#248046,#248047,#248048),(#248049,#248050,#248051),
(#248052,#248053,#248054),(#248055,#248056,#248057)),.UNSPECIFIED.,.F.,
 .F.,.F.)
B_SPLINE_SURFACE_WITH_KNOTS((4,4),(3,3),(-1.56938264467277E-17,0.000397394373651899),
(0.,1.),.UNSPECIFIED.)
GEOMETRIC_REPRESENTATION_ITEM()
RATIONAL_B_SPLINE_SURFACE(((1.,0.707106781186553,1.),(1.,0.707752587915868,
1.),(1.,0.708377654540695,1.),(1.,0.708689770883335,1.)))
REPRESENTATION_ITEM('')
SURFACE()
);
#3644=(
BOUNDED_SURFACE()
B_SPLINE_SURFACE(3,2,((#248059,#248060,#248061),(#248062,#248063,#248064),
(#248065,#248066,#248067),(#248068,#248069,#248070)),.UNSPECIFIED.,.F.,
 .F.,.F.)
B_SPLINE_SURFACE_WITH_KNOTS((4,4),(3,3),(-4.06575814682064E-19,0.000511815456479783),
(0.,1.0010587315981),.UNSPECIFIED.)
GEOMETRIC_REPRESENTATION_ITEM()
RATIONAL_B_SPLINE_SURFACE(((1.,0.708394529056873,1.00061746385253),(1.,
0.708058564167432,1.00061817524582),(1.,0.707430835372599,1.00061950443844),
(1.,0.706796685880911,1.00062084722665)))
REPRESENTATION_ITEM('')
SURFACE()
);
#3645=(
BOUNDED_SURFACE()
B_SPLINE_SURFACE(3,2,((#248076,#248077,#248078),(#248079,#248080,#248081),
(#248082,#248083,#248084),(#248085,#248086,#248087)),.UNSPECIFIED.,.F.,
 .F.,.F.)
B_SPLINE_SURFACE_WITH_KNOTS((4,4),(3,3),(-5.14996031930615E-19,0.000397394465448316),
(0.,1.),.UNSPECIFIED.)
GEOMETRIC_REPRESENTATION_ITEM()
RATIONAL_B_SPLINE_SURFACE(((1.,0.705498956110749,1.),(1.,0.705821764811784,
1.),(1.,0.70646195252115,1.),(1.,0.707106781186545,1.)))
REPRESENTATION_ITEM('')
SURFACE()
);
#3646=(
BOUNDED_SURFACE()
B_SPLINE_SURFACE(3,2,((#248093,#248094,#248095),(#248096,#248097,#248098),
(#248099,#248100,#248101),(#248102,#248103,#248104)),.UNSPECIFIED.,.F.,
 .F.,.F.)
B_SPLINE_SURFACE_WITH_KNOTS((4,4),(3,3),(5.96311194867027E-19,0.000397394410828733),
(0.,1.),.UNSPECIFIED.)
GEOMETRIC_REPRESENTATION_ITEM()
RATIONAL_B_SPLINE_SURFACE(((1.,0.708689770883335,1.),(1.,0.70837644003448,
1.),(1.,0.707750498698401,1.),(1.,0.70710678118655,1.)))
REPRESENTATION_ITEM('')
SURFACE()
);
#3647=(
BOUNDED_SURFACE()
B_SPLINE_SURFACE(3,2,((#248110,#248111,#248112),(#248113,#248114,#248115),
(#248116,#248117,#248118),(#248119,#248120,#248121)),.UNSPECIFIED.,.F.,
 .F.,.F.)
B_SPLINE_SURFACE_WITH_KNOTS((4,4),(3,3),(0.,0.000511815090126191),(0.,1.00105592270065),
 .UNSPECIFIED.)
GEOMETRIC_REPRESENTATION_ITEM()
RATIONAL_B_SPLINE_SURFACE(((1.,0.705266242717941,1.00062243212992),(1.,
0.705584085909598,1.00062176089424),(1.,0.706182089450967,1.00062049800321),
(1.,0.706797508587938,1.00061919833314)))
REPRESENTATION_ITEM('')
SURFACE()
);
#3648=(
BOUNDED_SURFACE()
B_SPLINE_SURFACE(3,2,((#248123,#248124,#248125),(#248126,#248127,#248128),
(#248129,#248130,#248131),(#248132,#248133,#248134)),.UNSPECIFIED.,.F.,
 .F.,.F.)
B_SPLINE_SURFACE_WITH_KNOTS((4,4),(3,3),(0.,0.000397394428086623),(0.,1.),
 .UNSPECIFIED.)
GEOMETRIC_REPRESENTATION_ITEM()
RATIONAL_B_SPLINE_SURFACE(((1.,0.70710678118655,1.),(1.,0.706459846759068,
1.),(1.,0.705820510737312,1.),(1.,0.70549895611075,1.)))
REPRESENTATION_ITEM('')
SURFACE()
);
#3649=(
BOUNDED_SURFACE()
B_SPLINE_SURFACE(3,2,((#248140,#248141,#248142),(#248143,#248144,#248145),
(#248146,#248147,#248148),(#248149,#248150,#248151),(#248152,#248153,#248154),
(#248155,#248156,#248157)),.UNSPECIFIED.,.F.,.F.,.F.)
B_SPLINE_SURFACE_WITH_KNOTS((4,2,4),(3,3),(0.,0.000257953807872843,0.000515907615745686),
(0.,1.),.UNSPECIFIED.)
GEOMETRIC_REPRESENTATION_ITEM()
RATIONAL_B_SPLINE_SURFACE(((1.,0.874619707139393,1.),(1.,0.874834349680018,
1.),(1.,0.85468610415643,1.),(1.,0.792476597916507,1.),(1.,0.750887854594091,
1.),(1.,0.705585838031455,1.)))
REPRESENTATION_ITEM('')
SURFACE()
);
#3650=(
BOUNDED_SURFACE()
B_SPLINE_SURFACE(3,2,((#248163,#248164,#248165),(#248166,#248167,#248168),
(#248169,#248170,#248171),(#248172,#248173,#248174)),.UNSPECIFIED.,.F.,
 .F.,.F.)
B_SPLINE_SURFACE_WITH_KNOTS((4,4),(3,3),(-8.13151629364128E-20,0.000511815437699164),
(0.,1.00105881331608),.UNSPECIFIED.)
GEOMETRIC_REPRESENTATION_ITEM()
RATIONAL_B_SPLINE_SURFACE(((1.,0.706796661946281,1.0006208951973),(1.,0.707430821225167,
1.00061955228472),(1.,0.70805854583067,1.00061822299838),(1.,0.708394505252657,
1.00061751156176)))
REPRESENTATION_ITEM('')
SURFACE()
);
#3651=(
BOUNDED_SURFACE()
B_SPLINE_SURFACE(3,2,((#248176,#248177,#248178),(#248179,#248180,#248181),
(#248182,#248183,#248184),(#248185,#248186,#248187),(#248188,#248189,#248190),
(#248191,#248192,#248193)),.UNSPECIFIED.,.F.,.F.,.F.)
B_SPLINE_SURFACE_WITH_KNOTS((4,2,4),(3,3),(-3.25260651745651E-19,0.000256915317531264,
0.000513830635062529),(0.,1.),.UNSPECIFIED.)
GEOMETRIC_REPRESENTATION_ITEM()
RATIONAL_B_SPLINE_SURFACE(((1.,0.70558583803144,1.),(1.,0.750902433542234,
1.),(1.,0.792329530083195,1.),(1.,0.854288401593536,1.),(1.,0.874998031125647,
1.),(1.,0.874619707139385,1.)))
REPRESENTATION_ITEM('')
SURFACE()
);
#3652=(
BOUNDED_SURFACE()
B_SPLINE_SURFACE(3,2,((#248199,#248200,#248201),(#248202,#248203,#248204),
(#248205,#248206,#248207),(#248208,#248209,#248210),(#248211,#248212,#248213),
(#248214,#248215,#248216)),.UNSPECIFIED.,.F.,.F.,.F.)
B_SPLINE_SURFACE_WITH_KNOTS((4,2,4),(3,3),(-3.6049722235143E-18,0.000256592814262163,
0.00051318562852433),(0.,1.),.UNSPECIFIED.)
GEOMETRIC_REPRESENTATION_ITEM()
RATIONAL_B_SPLINE_SURFACE(((1.,0.708712527163664,1.),(1.,0.753780902613515,
1.),(1.,0.794538995769305,1.),(1.,0.855070770331,1.),(1.,0.875018427445427,
1.),(1.,0.87461970713939,1.)))
REPRESENTATION_ITEM('')
SURFACE()
);
#3653=(
BOUNDED_SURFACE()
B_SPLINE_SURFACE(3,2,((#248218,#248219,#248220),(#248221,#248222,#248223),
(#248224,#248225,#248226),(#248227,#248228,#248229)),.UNSPECIFIED.,.F.,
 .F.,.F.)
B_SPLINE_SURFACE_WITH_KNOTS((4,4),(3,3),(-5.6920614055489E-19,0.000511815072430396),
(0.,1.00105598365828),.UNSPECIFIED.)
GEOMETRIC_REPRESENTATION_ITEM()
RATIONAL_B_SPLINE_SURFACE(((1.,0.706797490733857,1.0006192341167),(1.,0.706182062146763,
1.00062053388177),(1.,0.70558406276914,1.00062179683691),(1.,0.705266224770631,
1.00062246810037)))
REPRESENTATION_ITEM('')
SURFACE()
);
#3654=(
BOUNDED_SURFACE()
B_SPLINE_SURFACE(3,2,((#248235,#248236,#248237),(#248238,#248239,#248240),
(#248241,#248242,#248243),(#248244,#248245,#248246),(#248247,#248248,#248249),
(#248250,#248251,#248252)),.UNSPECIFIED.,.F.,.F.,.F.)
B_SPLINE_SURFACE_WITH_KNOTS((4,2,4),(3,3),(0.,0.000257652232350883,0.000515304464701766),
(0.,1.),.UNSPECIFIED.)
GEOMETRIC_REPRESENTATION_ITEM()
RATIONAL_B_SPLINE_SURFACE(((1.,0.874619707139399,1.),(1.,0.874861180430963,
1.),(1.,0.855455725920514,1.),(1.,0.794699358955633,1.),(1.,0.753768977788405,
1.),(1.,0.708712527163651,1.)))
REPRESENTATION_ITEM('')
SURFACE()
);
#3655=(
BOUNDED_SURFACE()
B_SPLINE_SURFACE(3,2,((#248258,#248259,#248260),(#248261,#248262,#248263),
(#248264,#248265,#248266),(#248267,#248268,#248269)),.UNSPECIFIED.,.F.,
 .F.,.F.)
B_SPLINE_SURFACE_WITH_KNOTS((4,4),(3,3),(0.,0.000397394373651917),(0.,1.),
 .UNSPECIFIED.)
GEOMETRIC_REPRESENTATION_ITEM()
RATIONAL_B_SPLINE_SURFACE(((1.,0.707106781186535,1.),(1.,0.707752587915927,
1.),(1.,0.708377654540653,1.),(1.,0.708689770883321,1.)))
REPRESENTATION_ITEM('')
SURFACE()
);
#3656=(
BOUNDED_SURFACE()
B_SPLINE_SURFACE(3,2,((#248271,#248272,#248273),(#248274,#248275,#248276),
(#248277,#248278,#248279),(#248280,#248281,#248282)),.UNSPECIFIED.,.F.,
 .F.,.F.)
B_SPLINE_SURFACE_WITH_KNOTS((4,4),(3,3),(0.,0.000511815456479791),(0.,1.00105873159918),
 .UNSPECIFIED.)
GEOMETRIC_REPRESENTATION_ITEM()
RATIONAL_B_SPLINE_SURFACE(((1.,0.708394529056554,1.00061746385316),(1.,
0.708058564167108,1.00061817524645),(1.,0.707430835372274,1.00061950443907),
(1.,0.70679668588061,1.00062084722729)))
REPRESENTATION_ITEM('')
SURFACE()
);
#3657=(
BOUNDED_SURFACE()
B_SPLINE_SURFACE(3,2,((#248288,#248289,#248290),(#248291,#248292,#248293),
(#248294,#248295,#248296),(#248297,#248298,#248299)),.UNSPECIFIED.,.F.,
 .F.,.F.)
B_SPLINE_SURFACE_WITH_KNOTS((4,4),(3,3),(-6.23416249179165E-19,0.000397394465448315),
(0.,1.),.UNSPECIFIED.)
GEOMETRIC_REPRESENTATION_ITEM()
RATIONAL_B_SPLINE_SURFACE(((1.,0.70549895611076,1.),(1.,0.705821764811773,
1.),(1.,0.706461952521134,1.),(1.,0.707106781186545,1.)))
REPRESENTATION_ITEM('')
SURFACE()
);
#3658=(
BOUNDED_SURFACE()
B_SPLINE_SURFACE(3,2,((#248305,#248306,#248307),(#248308,#248309,#248310),
(#248311,#248312,#248313),(#248314,#248315,#248316)),.UNSPECIFIED.,.F.,
 .F.,.F.)
B_SPLINE_SURFACE_WITH_KNOTS((4,4),(3,3),(0.,0.000397394410828731),(0.,1.),
 .UNSPECIFIED.)
GEOMETRIC_REPRESENTATION_ITEM()
RATIONAL_B_SPLINE_SURFACE(((1.,0.708689770883323,1.),(1.,0.708376440034482,
1.),(1.,0.707750498698435,1.),(1.,0.707106781186543,1.)))
REPRESENTATION_ITEM('')
SURFACE()
);
#3659=(
BOUNDED_SURFACE()
B_SPLINE_SURFACE(3,2,((#248322,#248323,#248324),(#248325,#248326,#248327),
(#248328,#248329,#248330),(#248331,#248332,#248333)),.UNSPECIFIED.,.F.,
 .F.,.F.)
B_SPLINE_SURFACE_WITH_KNOTS((4,4),(3,3),(0.,0.000511815090126181),(0.,1.00105592270032),
 .UNSPECIFIED.)
GEOMETRIC_REPRESENTATION_ITEM()
RATIONAL_B_SPLINE_SURFACE(((1.,0.705266242718053,1.00062243212973),(1.,
0.705584085909701,1.00062176089404),(1.,0.706182089451028,1.00062049800302),
(1.,0.706797508588036,1.00061919833294)))
REPRESENTATION_ITEM('')
SURFACE()
);
#3660=(
BOUNDED_SURFACE()
B_SPLINE_SURFACE(3,2,((#248335,#248336,#248337),(#248338,#248339,#248340),
(#248341,#248342,#248343),(#248344,#248345,#248346)),.UNSPECIFIED.,.F.,
 .F.,.F.)
B_SPLINE_SURFACE_WITH_KNOTS((4,4),(3,3),(0.,0.000397394428086633),(0.,1.),
 .UNSPECIFIED.)
GEOMETRIC_REPRESENTATION_ITEM()
RATIONAL_B_SPLINE_SURFACE(((1.,0.707106781186539,1.),(1.,0.706459846759122,
1.),(1.,0.705820510737294,1.),(1.,0.705498956110738,1.)))
REPRESENTATION_ITEM('')
SURFACE()
);
#3661=(
BOUNDED_SURFACE()
B_SPLINE_SURFACE(3,2,((#248352,#248353,#248354),(#248355,#248356,#248357),
(#248358,#248359,#248360),(#248361,#248362,#248363),(#248364,#248365,#248366),
(#248367,#248368,#248369)),.UNSPECIFIED.,.F.,.F.,.F.)
B_SPLINE_SURFACE_WITH_KNOTS((4,2,4),(3,3),(0.,0.000257953807872844,0.000515907615745689),
(0.,1.),.UNSPECIFIED.)
GEOMETRIC_REPRESENTATION_ITEM()
RATIONAL_B_SPLINE_SURFACE(((1.,0.874619707139397,1.),(1.,0.874834349679094,
1.),(1.,0.854686104157672,1.),(1.,0.792476597915231,1.),(1.,0.750887854595069,
1.),(1.,0.705585838031445,1.)))
REPRESENTATION_ITEM('')
SURFACE()
);
#3662=(
BOUNDED_SURFACE()
B_SPLINE_SURFACE(3,2,((#248375,#248376,#248377),(#248378,#248379,#248380),
(#248381,#248382,#248383),(#248384,#248385,#248386)),.UNSPECIFIED.,.F.,
 .F.,.F.)
B_SPLINE_SURFACE_WITH_KNOTS((4,4),(3,3),(5.6920614055489E-19,0.000511815437699151),
(0.,1.00105881331661),.UNSPECIFIED.)
GEOMETRIC_REPRESENTATION_ITEM()
RATIONAL_B_SPLINE_SURFACE(((1.,0.706796661946126,1.00062089519761),(1.,
0.707430821224996,1.00061955228503),(1.,0.708058545830506,1.00061822299869),
(1.,0.708394505252508,1.00061751156207)))
REPRESENTATION_ITEM('')
SURFACE()
);
#3663=(
BOUNDED_SURFACE()
B_SPLINE_SURFACE(3,2,((#248388,#248389,#248390),(#248391,#248392,#248393),
(#248394,#248395,#248396),(#248397,#248398,#248399),(#248400,#248401,#248402),
(#248403,#248404,#248405)),.UNSPECIFIED.,.F.,.F.,.F.)
B_SPLINE_SURFACE_WITH_KNOTS((4,2,4),(3,3),(0.,0.000256915317531267,0.000513830635062533),
(0.,1.),.UNSPECIFIED.)
GEOMETRIC_REPRESENTATION_ITEM()
RATIONAL_B_SPLINE_SURFACE(((1.,0.705585838031428,1.),(1.,0.750902433542297,
1.),(1.,0.792329530083163,1.),(1.,0.854288401593562,1.),(1.,0.874998031125636,
1.),(1.,0.874619707139394,1.)))
REPRESENTATION_ITEM('')
SURFACE()
);
#3664=(
BOUNDED_SURFACE()
B_SPLINE_SURFACE(3,2,((#248411,#248412,#248413),(#248414,#248415,#248416),
(#248417,#248418,#248419),(#248420,#248421,#248422),(#248423,#248424,#248425),
(#248426,#248427,#248428)),.UNSPECIFIED.,.F.,.F.,.F.)
B_SPLINE_SURFACE_WITH_KNOTS((4,2,4),(3,3),(-7.31836466427715E-19,0.000256592814262155,
0.000513185628524311),(0.,1.),.UNSPECIFIED.)
GEOMETRIC_REPRESENTATION_ITEM()
RATIONAL_B_SPLINE_SURFACE(((1.,0.708712527163665,1.),(1.,0.753780902613352,
1.),(1.,0.794538995769519,1.),(1.,0.855070770330792,1.),(1.,0.875018427445553,
1.),(1.,0.874619707139396,1.)))
REPRESENTATION_ITEM('')
SURFACE()
);
#3665=(
BOUNDED_SURFACE()
B_SPLINE_SURFACE(3,2,((#248430,#248431,#248432),(#248433,#248434,#248435),
(#248436,#248437,#248438),(#248439,#248440,#248441)),.UNSPECIFIED.,.F.,
 .F.,.F.)
B_SPLINE_SURFACE_WITH_KNOTS((4,4),(3,3),(0.,0.000511815072430391),(0.,1.00105598365643),
 .UNSPECIFIED.)
GEOMETRIC_REPRESENTATION_ITEM()
RATIONAL_B_SPLINE_SURFACE(((1.,0.706797490734398,1.00061923411562),(1.,
0.706182062147312,1.00062053388068),(1.,0.705584062769681,1.00062179683582),
(1.,0.705266224771159,1.00062246809928)))
REPRESENTATION_ITEM('')
SURFACE()
);
#3666=(
BOUNDED_SURFACE()
B_SPLINE_SURFACE(3,2,((#248447,#248448,#248449),(#248450,#248451,#248452),
(#248453,#248454,#248455),(#248456,#248457,#248458),(#248459,#248460,#248461),
(#248462,#248463,#248464)),.UNSPECIFIED.,.F.,.F.,.F.)
B_SPLINE_SURFACE_WITH_KNOTS((4,2,4),(3,3),(0.,0.000257652232350891,0.000515304464701781),
(0.,1.),.UNSPECIFIED.)
GEOMETRIC_REPRESENTATION_ITEM()
RATIONAL_B_SPLINE_SURFACE(((1.,0.874619707139387,1.),(1.,0.874861180430548,
1.),(1.,0.855455725921075,1.),(1.,0.794699358955069,1.),(1.,0.75376897778878,
1.),(1.,0.70871252716364,1.)))
REPRESENTATION_ITEM('')
SURFACE()
);
#3667=(
BOUNDED_SURFACE()
B_SPLINE_SURFACE(3,2,((#248470,#248471,#248472),(#248473,#248474,#248475),
(#248476,#248477,#248478),(#248479,#248480,#248481)),.UNSPECIFIED.,.F.,
 .F.,.F.)
B_SPLINE_SURFACE_WITH_KNOTS((4,4),(3,3),(-9.26992857475106E-18,0.000397394373651915),
(0.,1.),.UNSPECIFIED.)
GEOMETRIC_REPRESENTATION_ITEM()
RATIONAL_B_SPLINE_SURFACE(((1.,0.707106781186556,1.),(1.,0.707752587915886,
1.),(1.,0.708377654540688,1.),(1.,0.708689770883341,1.)))
REPRESENTATION_ITEM('')
SURFACE()
);
#3668=(
BOUNDED_SURFACE()
B_SPLINE_SURFACE(3,2,((#248483,#248484,#248485),(#248486,#248487,#248488),
(#248489,#248490,#248491),(#248492,#248493,#248494)),.UNSPECIFIED.,.F.,
 .F.,.F.)
B_SPLINE_SURFACE_WITH_KNOTS((4,4),(3,3),(0.,0.000511815456479786),(0.,1.00105873160137),
 .UNSPECIFIED.)
GEOMETRIC_REPRESENTATION_ITEM()
RATIONAL_B_SPLINE_SURFACE(((1.,0.708394529055883,1.00061746385444),(1.,
0.708058564166512,1.00061817524773),(1.,0.707430835371623,1.00061950444036),
(1.,0.706796685879971,1.00062084722857)))
REPRESENTATION_ITEM('')
SURFACE()
);
#3669=(
BOUNDED_SURFACE()
B_SPLINE_SURFACE(3,2,((#248500,#248501,#248502),(#248503,#248504,#248505),
(#248506,#248507,#248508),(#248509,#248510,#248511)),.UNSPECIFIED.,.F.,
 .F.,.F.)
B_SPLINE_SURFACE_WITH_KNOTS((4,4),(3,3),(-4.06575814682064E-18,0.000397394465448322),
(0.,1.),.UNSPECIFIED.)
GEOMETRIC_REPRESENTATION_ITEM()
RATIONAL_B_SPLINE_SURFACE(((1.,0.705498956110734,1.),(1.,0.70582176481179,
1.),(1.,0.706461952521119,1.),(1.,0.707106781186556,1.)))
REPRESENTATION_ITEM('')
SURFACE()
);
#3670=(
BOUNDED_SURFACE()
B_SPLINE_SURFACE(3,2,((#248517,#248518,#248519),(#248520,#248521,#248522),
(#248523,#248524,#248525),(#248526,#248527,#248528)),.UNSPECIFIED.,.F.,
 .F.,.F.)
B_SPLINE_SURFACE_WITH_KNOTS((4,4),(3,3),(0.,0.000397394410828732),(0.,1.),
 .UNSPECIFIED.)
GEOMETRIC_REPRESENTATION_ITEM()
RATIONAL_B_SPLINE_SURFACE(((1.,0.708689770883327,1.),(1.,0.708376440034498,
1.),(1.,0.707750498698427,1.),(1.,0.707106781186549,1.)))
REPRESENTATION_ITEM('')
SURFACE()
);
#3671=(
BOUNDED_SURFACE()
B_SPLINE_SURFACE(3,2,((#248534,#248535,#248536),(#248537,#248538,#248539),
(#248540,#248541,#248542),(#248543,#248544,#248545)),.UNSPECIFIED.,.F.,
 .F.,.F.)
B_SPLINE_SURFACE_WITH_KNOTS((4,4),(3,3),(-1.59919820441612E-18,0.000511815090126176),
(0.,1.00105592270011),.UNSPECIFIED.)
GEOMETRIC_REPRESENTATION_ITEM()
RATIONAL_B_SPLINE_SURFACE(((1.,0.705266242718087,1.0006224321296),(1.,0.705584085909776,
1.00062176089392),(1.,0.706182089451103,1.00062049800289),(1.,0.706797508588096,
1.00061919833282)))
REPRESENTATION_ITEM('')
SURFACE()
);
#3672=(
BOUNDED_SURFACE()
B_SPLINE_SURFACE(3,2,((#248547,#248548,#248549),(#248550,#248551,#248552),
(#248553,#248554,#248555),(#248556,#248557,#248558)),.UNSPECIFIED.,.F.,
 .F.,.F.)
B_SPLINE_SURFACE_WITH_KNOTS((4,4),(3,3),(0.,0.000397394428086635),(0.,1.),
 .UNSPECIFIED.)
GEOMETRIC_REPRESENTATION_ITEM()
RATIONAL_B_SPLINE_SURFACE(((1.,0.707106781186549,1.),(1.,0.706459846759078,
1.),(1.,0.705820510737299,1.),(1.,0.705498956110743,1.)))
REPRESENTATION_ITEM('')
SURFACE()
);
#3673=(
BOUNDED_SURFACE()
B_SPLINE_SURFACE(3,2,((#248564,#248565,#248566),(#248567,#248568,#248569),
(#248570,#248571,#248572),(#248573,#248574,#248575),(#248576,#248577,#248578),
(#248579,#248580,#248581)),.UNSPECIFIED.,.F.,.F.,.F.)
B_SPLINE_SURFACE_WITH_KNOTS((4,2,4),(3,3),(0.,0.000257953807872847,0.000515907615745694),
(0.,1.),.UNSPECIFIED.)
GEOMETRIC_REPRESENTATION_ITEM()
RATIONAL_B_SPLINE_SURFACE(((1.,0.874619707139385,1.),(1.,0.874834349678975,
1.),(1.,0.854686104157834,1.),(1.,0.792476597915104,1.),(1.,0.750887854595155,
1.),(1.,0.705585838031417,1.)))
REPRESENTATION_ITEM('')
SURFACE()
);
#3674=(
BOUNDED_SURFACE()
B_SPLINE_SURFACE(3,2,((#248587,#248588,#248589),(#248590,#248591,#248592),
(#248593,#248594,#248595),(#248596,#248597,#248598)),.UNSPECIFIED.,.F.,
 .F.,.F.)
B_SPLINE_SURFACE_WITH_KNOTS((4,4),(3,3),(0.,0.000511815437699152),(0.,1.00105881331622),
 .UNSPECIFIED.)
GEOMETRIC_REPRESENTATION_ITEM()
RATIONAL_B_SPLINE_SURFACE(((1.,0.706796661946239,1.00062089519738),(1.,
0.707430821225126,1.0006195522848),(1.,0.708058545830628,1.00061822299846),
(1.,0.708394505252628,1.00061751156184)))
REPRESENTATION_ITEM('')
SURFACE()
);
#3675=(
BOUNDED_SURFACE()
B_SPLINE_SURFACE(3,2,((#248600,#248601,#248602),(#248603,#248604,#248605),
(#248606,#248607,#248608),(#248609,#248610,#248611),(#248612,#248613,#248614),
(#248615,#248616,#248617)),.UNSPECIFIED.,.F.,.F.,.F.)
B_SPLINE_SURFACE_WITH_KNOTS((4,2,4),(3,3),(-8.6465123255719E-18,0.000256915317531255,
0.000513830635062519),(0.,1.),.UNSPECIFIED.)
GEOMETRIC_REPRESENTATION_ITEM()
RATIONAL_B_SPLINE_SURFACE(((1.,0.70558583803142,1.),(1.,0.750902433543074,
1.),(1.,0.792329530082077,1.),(1.,0.854288401594625,1.),(1.,0.874998031124799,
1.),(1.,0.874619707139392,1.)))
REPRESENTATION_ITEM('')
SURFACE()
);
#3676=(
BOUNDED_SURFACE()
B_SPLINE_SURFACE(3,2,((#248623,#248624,#248625),(#248626,#248627,#248628),
(#248629,#248630,#248631),(#248632,#248633,#248634),(#248635,#248636,#248637),
(#248638,#248639,#248640)),.UNSPECIFIED.,.F.,.F.,.F.)
B_SPLINE_SURFACE_WITH_KNOTS((4,2,4),(3,3),(-8.59230221694762E-18,0.000256592814262153,
0.000513185628524315),(0.,1.),.UNSPECIFIED.)
GEOMETRIC_REPRESENTATION_ITEM()
RATIONAL_B_SPLINE_SURFACE(((1.,0.708712527163675,1.),(1.,0.753780902613455,
1.),(1.,0.794538995769379,1.),(1.,0.855070770330912,1.),(1.,0.87501842744547,
1.),(1.,0.874619707139402,1.)))
REPRESENTATION_ITEM('')
SURFACE()
);
#3677=(
BOUNDED_SURFACE()
B_SPLINE_SURFACE(3,2,((#248642,#248643,#248644),(#248645,#248646,#248647),
(#248648,#248649,#248650),(#248651,#248652,#248653)),.UNSPECIFIED.,.F.,
 .F.,.F.)
B_SPLINE_SURFACE_WITH_KNOTS((4,4),(3,3),(0.,0.000511815072430396),(0.,1.00105598365749),
 .UNSPECIFIED.)
GEOMETRIC_REPRESENTATION_ITEM()
RATIONAL_B_SPLINE_SURFACE(((1.,0.706797490734088,1.00061923411624),(1.,
0.706182062147,1.0006205338813),(1.,0.705584062769387,1.00062179683644),
(1.,0.705266224770861,1.00062246809991)))
REPRESENTATION_ITEM('')
SURFACE()
);
#3678=(
BOUNDED_SURFACE()
B_SPLINE_SURFACE(3,2,((#248659,#248660,#248661),(#248662,#248663,#248664),
(#248665,#248666,#248667),(#248668,#248669,#248670),(#248671,#248672,#248673),
(#248674,#248675,#248676)),.UNSPECIFIED.,.F.,.F.,.F.)
B_SPLINE_SURFACE_WITH_KNOTS((4,2,4),(3,3),(-9.81202966099382E-18,0.000257652232350868,
0.000515304464701747),(0.,1.),.UNSPECIFIED.)
GEOMETRIC_REPRESENTATION_ITEM()
RATIONAL_B_SPLINE_SURFACE(((1.,0.874619707139399,1.),(1.,0.874861180430778,
1.),(1.,0.855455725920788,1.),(1.,0.794699358955341,1.),(1.,0.753768977788617,
1.),(1.,0.708712527163659,1.)))
REPRESENTATION_ITEM('')
SURFACE()
);
#3679=(
BOUNDED_SURFACE()
B_SPLINE_SURFACE(3,2,((#248682,#248683,#248684),(#248685,#248686,#248687),
(#248688,#248689,#248690),(#248691,#248692,#248693)),.UNSPECIFIED.,.F.,
 .F.,.F.)
B_SPLINE_SURFACE_WITH_KNOTS((4,4),(3,3),(5.96311194867027E-19,0.00039739437365192),
(0.,1.),.UNSPECIFIED.)
GEOMETRIC_REPRESENTATION_ITEM()
RATIONAL_B_SPLINE_SURFACE(((1.,0.707106781186546,1.),(1.,0.707752587915923,
1.),(1.,0.708377654540663,1.),(1.,0.708689770883323,1.)))
REPRESENTATION_ITEM('')
SURFACE()
);
#3680=(
BOUNDED_SURFACE()
B_SPLINE_SURFACE(3,2,((#248695,#248696,#248697),(#248698,#248699,#248700),
(#248701,#248702,#248703),(#248704,#248705,#248706)),.UNSPECIFIED.,.F.,
 .F.,.F.)
B_SPLINE_SURFACE_WITH_KNOTS((4,4),(3,3),(-1.62630325872826E-18,0.000511815456479784),
(0.,1.00105873160343),.UNSPECIFIED.)
GEOMETRIC_REPRESENTATION_ITEM()
RATIONAL_B_SPLINE_SURFACE(((1.,0.708394529055308,1.00061746385565),(1.,
0.708058564165876,1.00061817524894),(1.,0.707430835371038,1.00061950444157),
(1.,0.706796685879357,1.00062084722978)))
REPRESENTATION_ITEM('')
SURFACE()
);
#3681=(
BOUNDED_SURFACE()
B_SPLINE_SURFACE(3,2,((#248712,#248713,#248714),(#248715,#248716,#248717),
(#248718,#248719,#248720),(#248721,#248722,#248723)),.UNSPECIFIED.,.F.,
 .F.,.F.)
B_SPLINE_SURFACE_WITH_KNOTS((4,4),(3,3),(0.,0.0003973944654483),(0.,1.),
 .UNSPECIFIED.)
GEOMETRIC_REPRESENTATION_ITEM()
RATIONAL_B_SPLINE_SURFACE(((1.,0.705498956110752,1.),(1.,0.705821764811786,
1.),(1.,0.706461952521135,1.),(1.,0.707106781186546,1.)))
REPRESENTATION_ITEM('')
SURFACE()
);
#3682=(
BOUNDED_SURFACE()
B_SPLINE_SURFACE(3,2,((#248729,#248730,#248731),(#248732,#248733,#248734),
(#248735,#248736,#248737),(#248738,#248739,#248740)),.UNSPECIFIED.,.F.,
 .F.,.F.)
B_SPLINE_SURFACE_WITH_KNOTS((4,4),(3,3),(0.,0.00039739441082874),(0.,1.),
 .UNSPECIFIED.)
GEOMETRIC_REPRESENTATION_ITEM()
RATIONAL_B_SPLINE_SURFACE(((1.,0.708689770883324,1.),(1.,0.708376440034465,
1.),(1.,0.70775049869842,1.),(1.,0.707106781186549,1.)))
REPRESENTATION_ITEM('')
SURFACE()
);
#3683=(
BOUNDED_SURFACE()
B_SPLINE_SURFACE(3,2,((#248746,#248747,#248748),(#248749,#248750,#248751),
(#248752,#248753,#248754),(#248755,#248756,#248757)),.UNSPECIFIED.,.F.,
 .F.,.F.)
B_SPLINE_SURFACE_WITH_KNOTS((4,4),(3,3),(3.19839640883224E-18,0.000511815090126186),
(0.,1.00105592270213),.UNSPECIFIED.)
GEOMETRIC_REPRESENTATION_ITEM()
RATIONAL_B_SPLINE_SURFACE(((1.,0.705266242717516,1.0006224321308),(1.,0.705584085909153,
1.00062176089511),(1.,0.706182089450503,1.00062049800408),(1.,0.706797508587505,
1.00061919833401)))
REPRESENTATION_ITEM('')
SURFACE()
);
#3684=(
BOUNDED_SURFACE()
B_SPLINE_SURFACE(3,2,((#248759,#248760,#248761),(#248762,#248763,#248764),
(#248765,#248766,#248767),(#248768,#248769,#248770)),.UNSPECIFIED.,.F.,
 .F.,.F.)
B_SPLINE_SURFACE_WITH_KNOTS((4,4),(3,3),(-5.96311194867027E-19,0.000397394428086614),
(0.,1.),.UNSPECIFIED.)
GEOMETRIC_REPRESENTATION_ITEM()
RATIONAL_B_SPLINE_SURFACE(((1.,0.707106781186549,1.),(1.,0.70645984675909,
1.),(1.,0.705820510737294,1.),(1.,0.705498956110753,1.)))
REPRESENTATION_ITEM('')
SURFACE()
);
#3685=(
BOUNDED_SURFACE()
B_SPLINE_SURFACE(3,2,((#248776,#248777,#248778),(#248779,#248780,#248781),
(#248782,#248783,#248784),(#248785,#248786,#248787),(#248788,#248789,#248790),
(#248791,#248792,#248793)),.UNSPECIFIED.,.F.,.F.,.F.)
B_SPLINE_SURFACE_WITH_KNOTS((4,2,4),(3,3),(0.,0.000257953807872847,0.000515907615745694),
(0.,1.),.UNSPECIFIED.)
GEOMETRIC_REPRESENTATION_ITEM()
RATIONAL_B_SPLINE_SURFACE(((1.,0.874619707139392,1.),(1.,0.874834349678804,
1.),(1.,0.854686104158036,1.),(1.,0.792476597914902,1.),(1.,0.750887854595278,
1.),(1.,0.705585838031443,1.)))
REPRESENTATION_ITEM('')
SURFACE()
);
#3686=(
BOUNDED_SURFACE()
B_SPLINE_SURFACE(3,2,((#248799,#248800,#248801),(#248802,#248803,#248804),
(#248805,#248806,#248807),(#248808,#248809,#248810)),.UNSPECIFIED.,.F.,
 .F.,.F.)
B_SPLINE_SURFACE_WITH_KNOTS((4,4),(3,3),(-9.21571846612679E-18,0.000511815437699153),
(0.,1.00105881331631),.UNSPECIFIED.)
GEOMETRIC_REPRESENTATION_ITEM()
RATIONAL_B_SPLINE_SURFACE(((1.,0.706796661946213,1.00062089519743),(1.,
0.707430821225091,1.00061955228486),(1.,0.708058545830576,1.00061822299851),
(1.,0.70839450525259,1.00061751156189)))
REPRESENTATION_ITEM('')
SURFACE()
);
#3687=(
BOUNDED_SURFACE()
B_SPLINE_SURFACE(3,2,((#248812,#248813,#248814),(#248815,#248816,#248817),
(#248818,#248819,#248820),(#248821,#248822,#248823),(#248824,#248825,#248826),
(#248827,#248828,#248829)),.UNSPECIFIED.,.F.,.F.,.F.)
B_SPLINE_SURFACE_WITH_KNOTS((4,2,4),(3,3),(0.,0.000256915317531268,0.000513830635062536),
(0.,1.),.UNSPECIFIED.)
GEOMETRIC_REPRESENTATION_ITEM()
RATIONAL_B_SPLINE_SURFACE(((1.,0.705585838031433,1.),(1.,0.750902433542739,
1.),(1.,0.792329530082555,1.),(1.,0.854288401594177,1.),(1.,0.874998031125162,
1.),(1.,0.874619707139394,1.)))
REPRESENTATION_ITEM('')
SURFACE()
);
#3688=(
BOUNDED_SURFACE()
B_SPLINE_SURFACE(3,2,((#248835,#248836,#248837),(#248838,#248839,#248840),
(#248841,#248842,#248843),(#248844,#248845,#248846),(#248847,#248848,#248849),
(#248850,#248851,#248852)),.UNSPECIFIED.,.F.,.F.,.F.)
B_SPLINE_SURFACE_WITH_KNOTS((4,2,4),(3,3),(-1.43656787854329E-18,0.000256592814262153,
0.000513185628524308),(0.,1.),.UNSPECIFIED.)
GEOMETRIC_REPRESENTATION_ITEM()
RATIONAL_B_SPLINE_SURFACE(((1.,0.708712527163662,1.),(1.,0.75378090261378,
1.),(1.,0.794538995768932,1.),(1.,0.855070770331388,1.),(1.,0.87501842744511,
1.),(1.,0.874619707139403,1.)))
REPRESENTATION_ITEM('')
SURFACE()
);
#3689=(
BOUNDED_SURFACE()
B_SPLINE_SURFACE(3,2,((#248854,#248855,#248856),(#248857,#248858,#248859),
(#248860,#248861,#248862),(#248863,#248864,#248865)),.UNSPECIFIED.,.F.,
 .F.,.F.)
B_SPLINE_SURFACE_WITH_KNOTS((4,4),(3,3),(0.,0.000511815072430396),(0.,1.00105598365732),
 .UNSPECIFIED.)
GEOMETRIC_REPRESENTATION_ITEM()
RATIONAL_B_SPLINE_SURFACE(((1.,0.706797490734141,1.00061923411614),(1.,
0.706182062147035,1.0006205338812),(1.,0.705584062769417,1.00062179683634),
(1.,0.705266224770904,1.0006224680998)))
REPRESENTATION_ITEM('')
SURFACE()
);
#3690=(
BOUNDED_SURFACE()
B_SPLINE_SURFACE(3,2,((#248871,#248872,#248873),(#248874,#248875,#248876),
(#248877,#248878,#248879),(#248880,#248881,#248882),(#248883,#248884,#248885),
(#248886,#248887,#248888)),.UNSPECIFIED.,.F.,.F.,.F.)
B_SPLINE_SURFACE_WITH_KNOTS((4,2,4),(3,3),(-5.14996031930615E-19,0.00025765223235089,
0.000515304464701781),(0.,1.),.UNSPECIFIED.)
GEOMETRIC_REPRESENTATION_ITEM()
RATIONAL_B_SPLINE_SURFACE(((1.,0.874619707139388,1.),(1.,0.874861180431065,
1.),(1.,0.855455725920387,1.),(1.,0.794699358955754,1.),(1.,0.753768977788268,
1.),(1.,0.708712527163674,1.)))
REPRESENTATION_ITEM('')
SURFACE()
);
#3691=(
BOUNDED_SURFACE()
B_SPLINE_SURFACE(3,2,((#248894,#248895,#248896),(#248897,#248898,#248899),
(#248900,#248901,#248902),(#248903,#248904,#248905)),.UNSPECIFIED.,.F.,
 .F.,.F.)
B_SPLINE_SURFACE_WITH_KNOTS((4,4),(3,3),(0.,0.000397394373651913),(0.,1.),
 .UNSPECIFIED.)
GEOMETRIC_REPRESENTATION_ITEM()
RATIONAL_B_SPLINE_SURFACE(((1.,0.707106781186546,1.),(1.,0.707752587915897,
1.),(1.,0.708377654540679,1.),(1.,0.708689770883326,1.)))
REPRESENTATION_ITEM('')
SURFACE()
);
#3692=(
BOUNDED_SURFACE()
B_SPLINE_SURFACE(3,2,((#248907,#248908,#248909),(#248910,#248911,#248912),
(#248913,#248914,#248915),(#248916,#248917,#248918)),.UNSPECIFIED.,.F.,
 .F.,.F.)
B_SPLINE_SURFACE_WITH_KNOTS((4,4),(3,3),(0.,0.000511815456479785),(0.,1.00105873159871),
 .UNSPECIFIED.)
GEOMETRIC_REPRESENTATION_ITEM()
RATIONAL_B_SPLINE_SURFACE(((1.,0.708394529056685,1.00061746385289),(1.,
0.708058564167261,1.00061817524618),(1.,0.70743083537241,1.0006195044388),
(1.,0.706796685880754,1.00062084722701)))
REPRESENTATION_ITEM('')
SURFACE()
);
#3693=(
BOUNDED_SURFACE()
B_SPLINE_SURFACE(3,2,((#248924,#248925,#248926),(#248927,#248928,#248929),
(#248930,#248931,#248932),(#248933,#248934,#248935)),.UNSPECIFIED.,.F.,
 .F.,.F.)
B_SPLINE_SURFACE_WITH_KNOTS((4,4),(3,3),(0.,0.000397394465448299),(0.,1.),
 .UNSPECIFIED.)
GEOMETRIC_REPRESENTATION_ITEM()
RATIONAL_B_SPLINE_SURFACE(((1.,0.705498956110716,1.),(1.,0.705821764811794,
1.),(1.,0.706461952521151,1.),(1.,0.707106781186533,1.)))
REPRESENTATION_ITEM('')
SURFACE()
);
#3694=(
BOUNDED_SURFACE()
B_SPLINE_SURFACE(3,2,((#248941,#248942,#248943),(#248944,#248945,#248946),
(#248947,#248948,#248949),(#248950,#248951,#248952)),.UNSPECIFIED.,.F.,
 .F.,.F.)
B_SPLINE_SURFACE_WITH_KNOTS((4,4),(3,3),(0.,0.000397394410828737),(0.,1.),
 .UNSPECIFIED.)
GEOMETRIC_REPRESENTATION_ITEM()
RATIONAL_B_SPLINE_SURFACE(((1.,0.708689770883333,1.),(1.,0.708376440034488,
1.),(1.,0.7077504986984,1.),(1.,0.70710678118656,1.)))
REPRESENTATION_ITEM('')
SURFACE()
);
#3695=(
BOUNDED_SURFACE()
B_SPLINE_SURFACE(3,2,((#248958,#248959,#248960),(#248961,#248962,#248963),
(#248964,#248965,#248966),(#248967,#248968,#248969)),.UNSPECIFIED.,.F.,
 .F.,.F.)
B_SPLINE_SURFACE_WITH_KNOTS((4,4),(3,3),(0.,0.00051181509012619),(0.,1.00105592269933),
 .UNSPECIFIED.)
GEOMETRIC_REPRESENTATION_ITEM()
RATIONAL_B_SPLINE_SURFACE(((1.,0.705266242718325,1.00062243212914),(1.,
0.705584085909984,1.00062176089346),(1.,0.70618208945133,1.00062049800243),
(1.,0.706797508588325,1.00061919833236)))
REPRESENTATION_ITEM('')
SURFACE()
);
#3696=(
BOUNDED_SURFACE()
B_SPLINE_SURFACE(3,2,((#248971,#248972,#248973),(#248974,#248975,#248976),
(#248977,#248978,#248979),(#248980,#248981,#248982)),.UNSPECIFIED.,.F.,
 .F.,.F.)
B_SPLINE_SURFACE_WITH_KNOTS((4,4),(3,3),(-6.26126754610379E-18,0.000397394428086626),
(0.,1.),.UNSPECIFIED.)
GEOMETRIC_REPRESENTATION_ITEM()
RATIONAL_B_SPLINE_SURFACE(((1.,0.707106781186549,1.),(1.,0.706459846759093,
1.),(1.,0.705820510737289,1.),(1.,0.705498956110746,1.)))
REPRESENTATION_ITEM('')
SURFACE()
);
#3697=(
BOUNDED_SURFACE()
B_SPLINE_SURFACE(3,2,((#248988,#248989,#248990),(#248991,#248992,#248993),
(#248994,#248995,#248996),(#248997,#248998,#248999),(#249000,#249001,#249002),
(#249003,#249004,#249005)),.UNSPECIFIED.,.F.,.F.,.F.)
B_SPLINE_SURFACE_WITH_KNOTS((4,2,4),(3,3),(0.,0.000257953807872849,0.000515907615745697),
(0.,1.),.UNSPECIFIED.)
GEOMETRIC_REPRESENTATION_ITEM()
RATIONAL_B_SPLINE_SURFACE(((1.,0.874619707139393,1.),(1.,0.874834349679035,
1.),(1.,0.854686104157749,1.),(1.,0.792476597915191,1.),(1.,0.750887854595084,
1.),(1.,0.705585838031438,1.)))
REPRESENTATION_ITEM('')
SURFACE()
);
#3698=(
BOUNDED_SURFACE()
B_SPLINE_SURFACE(3,2,((#249011,#249012,#249013),(#249014,#249015,#249016),
(#249017,#249018,#249019),(#249020,#249021,#249022)),.UNSPECIFIED.,.F.,
 .F.,.F.)
B_SPLINE_SURFACE_WITH_KNOTS((4,4),(3,3),(0.,0.00051181543769915),(0.,1.00105881331638),
 .UNSPECIFIED.)
GEOMETRIC_REPRESENTATION_ITEM()
RATIONAL_B_SPLINE_SURFACE(((1.,0.706796661946193,1.00062089519747),(1.,
0.707430821225081,1.0006195522849),(1.,0.708058545830556,1.00061822299855),
(1.,0.708394505252586,1.00061751156193)))
REPRESENTATION_ITEM('')
SURFACE()
);
#3699=(
BOUNDED_SURFACE()
B_SPLINE_SURFACE(3,2,((#249024,#249025,#249026),(#249027,#249028,#249029),
(#249030,#249031,#249032),(#249033,#249034,#249035),(#249036,#249037,#249038),
(#249039,#249040,#249041)),.UNSPECIFIED.,.F.,.F.,.F.)
B_SPLINE_SURFACE_WITH_KNOTS((4,2,4),(3,3),(2.90024081139872E-18,0.000256915317531264,
0.000513830635062526),(0.,1.),.UNSPECIFIED.)
GEOMETRIC_REPRESENTATION_ITEM()
RATIONAL_B_SPLINE_SURFACE(((1.,0.705585838031437,1.),(1.,0.750902433543791,
1.),(1.,0.792329530081131,1.),(1.,0.854288401595599,1.),(1.,0.874998031124076,
1.),(1.,0.874619707139391,1.)))
REPRESENTATION_ITEM('')
SURFACE()
);
#3700=(
BOUNDED_SURFACE()
B_SPLINE_SURFACE(3,2,((#249047,#249048,#249049),(#249050,#249051,#249052),
(#249053,#249054,#249055),(#249056,#249057,#249058),(#249059,#249060,#249061),
(#249062,#249063,#249064)),.UNSPECIFIED.,.F.,.F.,.F.)
B_SPLINE_SURFACE_WITH_KNOTS((4,2,4),(3,3),(0.,0.000256592814262157,0.000513185628524314),
(0.,1.),.UNSPECIFIED.)
GEOMETRIC_REPRESENTATION_ITEM()
RATIONAL_B_SPLINE_SURFACE(((1.,0.708712527163633,1.),(1.,0.753780902613117,
1.),(1.,0.794538995769877,1.),(1.,0.855070770330416,1.),(1.,0.875018427445846,
1.),(1.,0.874619707139403,1.)))
REPRESENTATION_ITEM('')
SURFACE()
);
#3701=(
BOUNDED_SURFACE()
B_SPLINE_SURFACE(3,2,((#249066,#249067,#249068),(#249069,#249070,#249071),
(#249072,#249073,#249074),(#249075,#249076,#249077)),.UNSPECIFIED.,.F.,
 .F.,.F.)
B_SPLINE_SURFACE_WITH_KNOTS((4,4),(3,3),(0.,0.000511815072430398),(0.,1.00105598365789),
 .UNSPECIFIED.)
GEOMETRIC_REPRESENTATION_ITEM()
RATIONAL_B_SPLINE_SURFACE(((1.,0.706797490733974,1.00061923411647),(1.,
0.706182062146914,1.00062053388153),(1.,0.705584062769252,1.00062179683667),
(1.,0.705266224770738,1.00062246810014)))
REPRESENTATION_ITEM('')
SURFACE()
);
#3702=(
BOUNDED_SURFACE()
B_SPLINE_SURFACE(3,2,((#249083,#249084,#249085),(#249086,#249087,#249088),
(#249089,#249090,#249091),(#249092,#249093,#249094),(#249095,#249096,#249097),
(#249098,#249099,#249100)),.UNSPECIFIED.,.F.,.F.,.F.)
B_SPLINE_SURFACE_WITH_KNOTS((4,2,4),(3,3),(0.,0.000257652232350886,0.000515304464701772),
(0.,1.),.UNSPECIFIED.)
GEOMETRIC_REPRESENTATION_ITEM()
RATIONAL_B_SPLINE_SURFACE(((1.,0.874619707139397,1.),(1.,0.874861180430422,
1.),(1.,0.855455725921253,1.),(1.,0.794699358954883,1.),(1.,0.753768977788929,
1.),(1.,0.708712527163669,1.)))
REPRESENTATION_ITEM('')
SURFACE()
);
#3703=(
BOUNDED_SURFACE()
B_SPLINE_SURFACE(3,2,((#249106,#249107,#249108),(#249109,#249110,#249111),
(#249112,#249113,#249114),(#249115,#249116,#249117)),.UNSPECIFIED.,.F.,
 .F.,.F.)
B_SPLINE_SURFACE_WITH_KNOTS((4,4),(3,3),(0.,0.000397394373651908),(0.,1.),
 .UNSPECIFIED.)
GEOMETRIC_REPRESENTATION_ITEM()
RATIONAL_B_SPLINE_SURFACE(((1.,0.707106781186546,1.),(1.,0.707752587915901,
1.),(1.,0.708377654540672,1.),(1.,0.708689770883331,1.)))
REPRESENTATION_ITEM('')
SURFACE()
);
#3704=(
BOUNDED_SURFACE()
B_SPLINE_SURFACE(3,2,((#249119,#249120,#249121),(#249122,#249123,#249124),
(#249125,#249126,#249127),(#249128,#249129,#249130)),.UNSPECIFIED.,.F.,
 .F.,.F.)
B_SPLINE_SURFACE_WITH_KNOTS((4,4),(3,3),(0.,0.000511815456479783),(0.,1.00105873160032),
 .UNSPECIFIED.)
GEOMETRIC_REPRESENTATION_ITEM()
RATIONAL_B_SPLINE_SURFACE(((1.,0.708394529056214,1.00061746385383),(1.,
0.70805856416676,1.00061817524712),(1.,0.707430835371966,1.00061950443974),
(1.,0.706796685880259,1.00062084722795)))
REPRESENTATION_ITEM('')
SURFACE()
);
#3705=(
BOUNDED_SURFACE()
B_SPLINE_SURFACE(3,2,((#249136,#249137,#249138),(#249139,#249140,#249141),
(#249142,#249143,#249144),(#249145,#249146,#249147)),.UNSPECIFIED.,.F.,
 .F.,.F.)
B_SPLINE_SURFACE_WITH_KNOTS((4,4),(3,3),(0.,0.000397394465448303),(0.,1.),
 .UNSPECIFIED.)
GEOMETRIC_REPRESENTATION_ITEM()
RATIONAL_B_SPLINE_SURFACE(((1.,0.705498956110751,1.),(1.,0.705821764811794,
1.),(1.,0.706461952521126,1.),(1.,0.707106781186546,1.)))
REPRESENTATION_ITEM('')
SURFACE()
);
#3706=(
BOUNDED_SURFACE()
B_SPLINE_SURFACE(3,2,((#249153,#249154,#249155),(#249156,#249157,#249158),
(#249159,#249160,#249161),(#249162,#249163,#249164)),.UNSPECIFIED.,.F.,
 .F.,.F.)
B_SPLINE_SURFACE_WITH_KNOTS((4,4),(3,3),(0.,0.000397394410828739),(0.,1.),
 .UNSPECIFIED.)
GEOMETRIC_REPRESENTATION_ITEM()
RATIONAL_B_SPLINE_SURFACE(((1.,0.708689770883341,1.),(1.,0.708376440034498,
1.),(1.,0.707750498698416,1.),(1.,0.70710678118655,1.)))
REPRESENTATION_ITEM('')
SURFACE()
);
#3707=(
BOUNDED_SURFACE()
B_SPLINE_SURFACE(3,2,((#249170,#249171,#249172),(#249173,#249174,#249175),
(#249176,#249177,#249178),(#249179,#249180,#249181)),.UNSPECIFIED.,.F.,
 .F.,.F.)
B_SPLINE_SURFACE_WITH_KNOTS((4,4),(3,3),(-4.06575814682064E-19,0.000511815090126176),
(0.,1.00105592270253),.UNSPECIFIED.)
GEOMETRIC_REPRESENTATION_ITEM()
RATIONAL_B_SPLINE_SURFACE(((1.,0.705266242717368,1.00062243213103),(1.,
0.705584085909073,1.00062176089535),(1.,0.706182089450375,1.00062049800432),
(1.,0.706797508587387,1.00061919833424)))
REPRESENTATION_ITEM('')
SURFACE()
);
#3708=(
BOUNDED_SURFACE()
B_SPLINE_SURFACE(3,2,((#249183,#249184,#249185),(#249186,#249187,#249188),
(#249189,#249190,#249191),(#249192,#249193,#249194)),.UNSPECIFIED.,.F.,
 .F.,.F.)
B_SPLINE_SURFACE_WITH_KNOTS((4,4),(3,3),(-5.42101086242752E-20,0.000397394428086623),
(0.,1.),.UNSPECIFIED.)
GEOMETRIC_REPRESENTATION_ITEM()
RATIONAL_B_SPLINE_SURFACE(((1.,0.707106781186549,1.),(1.,0.706459846759087,
1.),(1.,0.705820510737284,1.),(1.,0.705498956110736,1.)))
REPRESENTATION_ITEM('')
SURFACE()
);
#3709=(
BOUNDED_SURFACE()
B_SPLINE_SURFACE(3,2,((#249200,#249201,#249202),(#249203,#249204,#249205),
(#249206,#249207,#249208),(#249209,#249210,#249211),(#249212,#249213,#249214),
(#249215,#249216,#249217)),.UNSPECIFIED.,.F.,.F.,.F.)
B_SPLINE_SURFACE_WITH_KNOTS((4,2,4),(3,3),(0.,0.000257953807872845,0.00051590761574569),
(0.,1.),.UNSPECIFIED.)
GEOMETRIC_REPRESENTATION_ITEM()
RATIONAL_B_SPLINE_SURFACE(((1.,0.874619707139394,1.),(1.,0.874834349679555,
1.),(1.,0.854686104157056,1.),(1.,0.792476597915864,1.),(1.,0.750887854594591,
1.),(1.,0.705585838031442,1.)))
REPRESENTATION_ITEM('')
SURFACE()
);
#3710=(
BOUNDED_SURFACE()
B_SPLINE_SURFACE(3,2,((#249223,#249224,#249225),(#249226,#249227,#249228),
(#249229,#249230,#249231),(#249232,#249233,#249234)),.UNSPECIFIED.,.F.,
 .F.,.F.)
B_SPLINE_SURFACE_WITH_KNOTS((4,4),(3,3),(0.,0.00051181543769915),(0.,1.00105881331787),
 .UNSPECIFIED.)
GEOMETRIC_REPRESENTATION_ITEM()
RATIONAL_B_SPLINE_SURFACE(((1.,0.706796661945757,1.00062089519835),(1.,
0.707430821224658,1.00061955228577),(1.,0.708058545830111,1.00061822299943),
(1.,0.708394505252165,1.00061751156281)))
REPRESENTATION_ITEM('')
SURFACE()
);
#3711=(
BOUNDED_SURFACE()
B_SPLINE_SURFACE(3,2,((#249236,#249237,#249238),(#249239,#249240,#249241),
(#249242,#249243,#249244),(#249245,#249246,#249247),(#249248,#249249,#249250),
(#249251,#249252,#249253)),.UNSPECIFIED.,.F.,.F.,.F.)
B_SPLINE_SURFACE_WITH_KNOTS((4,2,4),(3,3),(0.,0.000256915317531267,0.000513830635062535),
(0.,1.),.UNSPECIFIED.)
GEOMETRIC_REPRESENTATION_ITEM()
RATIONAL_B_SPLINE_SURFACE(((1.,0.705585838031432,1.),(1.,0.750902433542741,
1.),(1.,0.792329530082537,1.),(1.,0.854288401594207,1.),(1.,0.874998031125139,
1.),(1.,0.874619707139396,1.)))
REPRESENTATION_ITEM('')
SURFACE()
);
#3712=(
BOUNDED_SURFACE()
B_SPLINE_SURFACE(3,2,((#249259,#249260,#249261),(#249262,#249263,#249264),
(#249265,#249266,#249267),(#249268,#249269,#249270),(#249271,#249272,#249273),
(#249274,#249275,#249276)),.UNSPECIFIED.,.F.,.F.,.F.)
B_SPLINE_SURFACE_WITH_KNOTS((4,2,4),(3,3),(-2.87313575708659E-18,0.000256592814262152,
0.000513185628524308),(0.,1.),.UNSPECIFIED.)
GEOMETRIC_REPRESENTATION_ITEM()
RATIONAL_B_SPLINE_SURFACE(((1.,0.708712527163668,1.),(1.,0.753780902614103,
1.),(1.,0.79453899576851,1.),(1.,0.855070770331806,1.),(1.,0.875018427444798,
1.),(1.,0.874619707139392,1.)))
REPRESENTATION_ITEM('')
SURFACE()
);
#3713=(
BOUNDED_SURFACE()
B_SPLINE_SURFACE(3,2,((#249278,#249279,#249280),(#249281,#249282,#249283),
(#249284,#249285,#249286),(#249287,#249288,#249289)),.UNSPECIFIED.,.F.,
 .F.,.F.)
B_SPLINE_SURFACE_WITH_KNOTS((4,4),(3,3),(0.,0.000511815072430403),(0.,1.00105598365859),
 .UNSPECIFIED.)
GEOMETRIC_REPRESENTATION_ITEM()
RATIONAL_B_SPLINE_SURFACE(((1.,0.706797490733767,1.00061923411689),(1.,
0.706182062146727,1.00062053388195),(1.,0.705584062769004,1.00062179683709),
(1.,0.705266224770526,1.00062246810056)))
REPRESENTATION_ITEM('')
SURFACE()
);
#3714=(
BOUNDED_SURFACE()
B_SPLINE_SURFACE(3,2,((#249295,#249296,#249297),(#249298,#249299,#249300),
(#249301,#249302,#249303),(#249304,#249305,#249306),(#249307,#249308,#249309),
(#249310,#249311,#249312)),.UNSPECIFIED.,.F.,.F.,.F.)
B_SPLINE_SURFACE_WITH_KNOTS((4,2,4),(3,3),(-2.87313575708659E-18,0.000257652232350883,
0.000515304464701769),(0.,1.),.UNSPECIFIED.)
GEOMETRIC_REPRESENTATION_ITEM()
RATIONAL_B_SPLINE_SURFACE(((1.,0.874619707139394,1.),(1.,0.874861180430723,
1.),(1.,0.85545572592083,1.),(1.,0.794699358955305,1.),(1.,0.753768977788583,
1.),(1.,0.708712527163669,1.)))
REPRESENTATION_ITEM('')
SURFACE()
);
#3715=(
BOUNDED_SURFACE()
B_SPLINE_SURFACE(3,2,((#249318,#249319,#249320),(#249321,#249322,#249323),
(#249324,#249325,#249326),(#249327,#249328,#249329)),.UNSPECIFIED.,.F.,
 .F.,.F.)
B_SPLINE_SURFACE_WITH_KNOTS((4,4),(3,3),(-7.86046575051991E-18,0.000397394373651897),
(0.,1.),.UNSPECIFIED.)
GEOMETRIC_REPRESENTATION_ITEM()
RATIONAL_B_SPLINE_SURFACE(((1.,0.707106781186546,1.),(1.,0.707752587915903,
1.),(1.,0.708377654540693,1.),(1.,0.708689770883325,1.)))
REPRESENTATION_ITEM('')
SURFACE()
);
#3716=(
BOUNDED_SURFACE()
B_SPLINE_SURFACE(3,2,((#249331,#249332,#249333),(#249334,#249335,#249336),
(#249337,#249338,#249339),(#249340,#249341,#249342)),.UNSPECIFIED.,.F.,
 .F.,.F.)
B_SPLINE_SURFACE_WITH_KNOTS((4,4),(3,3),(0.,0.000511815456479783),(0.,1.00105873160118),
 .UNSPECIFIED.)
GEOMETRIC_REPRESENTATION_ITEM()
RATIONAL_B_SPLINE_SURFACE(((1.,0.708394529055962,1.00061746385433),(1.,
0.708058564166525,1.00061817524762),(1.,0.707430835371686,1.00061950444025),
(1.,0.706796685880017,1.00062084722846)))
REPRESENTATION_ITEM('')
SURFACE()
);
#3717=(
BOUNDED_SURFACE()
B_SPLINE_SURFACE(3,2,((#249348,#249349,#249350),(#249351,#249352,#249353),
(#249354,#249355,#249356),(#249357,#249358,#249359)),.UNSPECIFIED.,.F.,
 .F.,.F.)
B_SPLINE_SURFACE_WITH_KNOTS((4,4),(3,3),(-6.09863722023096E-18,0.000397394465448312),
(0.,1.),.UNSPECIFIED.)
GEOMETRIC_REPRESENTATION_ITEM()
RATIONAL_B_SPLINE_SURFACE(((1.,0.705498956110748,1.),(1.,0.705821764811799,
1.),(1.,0.706461952521121,1.),(1.,0.707106781186555,1.)))
REPRESENTATION_ITEM('')
SURFACE()
);
#3718=(
BOUNDED_SURFACE()
B_SPLINE_SURFACE(3,2,((#249365,#249366,#249367),(#249368,#249369,#249370),
(#249371,#249372,#249373),(#249374,#249375,#249376)),.UNSPECIFIED.,.F.,
 .F.,.F.)
B_SPLINE_SURFACE_WITH_KNOTS((4,4),(3,3),(0.,0.000397394410828749),(0.,1.),
 .UNSPECIFIED.)
GEOMETRIC_REPRESENTATION_ITEM()
RATIONAL_B_SPLINE_SURFACE(((1.,0.708689770883337,1.),(1.,0.708376440034518,
1.),(1.,0.707750498698402,1.),(1.,0.707106781186549,1.)))
REPRESENTATION_ITEM('')
SURFACE()
);
#3719=(
BOUNDED_SURFACE()
B_SPLINE_SURFACE(3,2,((#249382,#249383,#249384),(#249385,#249386,#249387),
(#249388,#249389,#249390),(#249391,#249392,#249393)),.UNSPECIFIED.,.F.,
 .F.,.F.)
B_SPLINE_SURFACE_WITH_KNOTS((4,4),(3,3),(-5.23127548224256E-18,0.000511815090126196),
(0.,1.00105592270209),.UNSPECIFIED.)
GEOMETRIC_REPRESENTATION_ITEM()
RATIONAL_B_SPLINE_SURFACE(((1.,0.705266242717518,1.00062243213078),(1.,
0.705584085909157,1.00062176089509),(1.,0.706182089450553,1.00062049800406),
(1.,0.706797508587506,1.00061919833399)))
REPRESENTATION_ITEM('')
SURFACE()
);
#3720=(
BOUNDED_SURFACE()
B_SPLINE_SURFACE(3,2,((#249395,#249396,#249397),(#249398,#249399,#249400),
(#249401,#249402,#249403),(#249404,#249405,#249406)),.UNSPECIFIED.,.F.,
 .F.,.F.)
B_SPLINE_SURFACE_WITH_KNOTS((4,4),(3,3),(-5.6920614055489E-19,0.000397394428086642),
(0.,1.),.UNSPECIFIED.)
GEOMETRIC_REPRESENTATION_ITEM()
RATIONAL_B_SPLINE_SURFACE(((1.,0.707106781186549,1.),(1.,0.706459846759097,
1.),(1.,0.705820510737282,1.),(1.,0.705498956110751,1.)))
REPRESENTATION_ITEM('')
SURFACE()
);
#3721=(
BOUNDED_SURFACE()
B_SPLINE_SURFACE(3,2,((#249412,#249413,#249414),(#249415,#249416,#249417),
(#249418,#249419,#249420),(#249421,#249422,#249423),(#249424,#249425,#249426),
(#249427,#249428,#249429)),.UNSPECIFIED.,.F.,.F.,.F.)
B_SPLINE_SURFACE_WITH_KNOTS((4,2,4),(3,3),(0.,0.000257953807872837,0.000515907615745674),
(0.,1.),.UNSPECIFIED.)
GEOMETRIC_REPRESENTATION_ITEM()
RATIONAL_B_SPLINE_SURFACE(((1.,0.874619707139396,1.),(1.,0.87483434967922,
1.),(1.,0.854686104157491,1.),(1.,0.792476597915446,1.),(1.,0.750887854594912,
1.),(1.,0.705585838031434,1.)))
REPRESENTATION_ITEM('')
SURFACE()
);
#3722=(
BOUNDED_SURFACE()
B_SPLINE_SURFACE(3,2,((#249435,#249436,#249437),(#249438,#249439,#249440),
(#249441,#249442,#249443),(#249444,#249445,#249446)),.UNSPECIFIED.,.F.,
 .F.,.F.)
B_SPLINE_SURFACE_WITH_KNOTS((4,4),(3,3),(0.,0.00051181543769915),(0.,1.00105881331998),
 .UNSPECIFIED.)
GEOMETRIC_REPRESENTATION_ITEM()
RATIONAL_B_SPLINE_SURFACE(((1.,0.706796661945137,1.00062089519959),(1.,
0.707430821224013,1.00061955228701),(1.,0.708058545829528,1.00061822300066),
(1.,0.708394505251531,1.00061751156404)))
REPRESENTATION_ITEM('')
SURFACE()
);
#3723=(
BOUNDED_SURFACE()
B_SPLINE_SURFACE(3,2,((#249448,#249449,#249450),(#249451,#249452,#249453),
(#249454,#249455,#249456),(#249457,#249458,#249459),(#249460,#249461,#249462),
(#249463,#249464,#249465)),.UNSPECIFIED.,.F.,.F.,.F.)
B_SPLINE_SURFACE_WITH_KNOTS((4,2,4),(3,3),(0.,0.000256915317531263,0.000513830635062527),
(0.,1.),.UNSPECIFIED.)
GEOMETRIC_REPRESENTATION_ITEM()
RATIONAL_B_SPLINE_SURFACE(((1.,0.705585838031439,1.),(1.,0.750902433542964,
1.),(1.,0.792329530082284,1.),(1.,0.854288401594488,1.),(1.,0.874998031124956,
1.),(1.,0.874619707139399,1.)))
REPRESENTATION_ITEM('')
SURFACE()
);
#3724=(
BOUNDED_SURFACE()
B_SPLINE_SURFACE(3,2,((#249471,#249472,#249473),(#249474,#249475,#249476),
(#249477,#249478,#249479),(#249480,#249481,#249482),(#249483,#249484,#249485),
(#249486,#249487,#249488)),.UNSPECIFIED.,.F.,.F.,.F.)
B_SPLINE_SURFACE_WITH_KNOTS((4,2,4),(3,3),(-1.81603863891322E-18,0.000256592814262153,
0.000513185628524309),(0.,1.),.UNSPECIFIED.)
GEOMETRIC_REPRESENTATION_ITEM()
RATIONAL_B_SPLINE_SURFACE(((1.,0.708712527163673,1.),(1.,0.753780902614018,
1.),(1.,0.794538995768624,1.),(1.,0.855070770331673,1.),(1.,0.875018427444898,
1.),(1.,0.8746197071394,1.)))
REPRESENTATION_ITEM('')
SURFACE()
);
#3725=(
BOUNDED_SURFACE()
B_SPLINE_SURFACE(3,2,((#249490,#249491,#249492),(#249493,#249494,#249495),
(#249496,#249497,#249498),(#249499,#249500,#249501)),.UNSPECIFIED.,.F.,
 .F.,.F.)
B_SPLINE_SURFACE_WITH_KNOTS((4,4),(3,3),(-2.71050543121376E-20,0.00051181507243041),
(0.,1.00105598366023),.UNSPECIFIED.)
GEOMETRIC_REPRESENTATION_ITEM()
RATIONAL_B_SPLINE_SURFACE(((1.,0.706797490733287,1.00061923411785),(1.,
0.706182062146206,1.00062053388291),(1.,0.705584062768565,1.00062179683806),
(1.,0.705266224770061,1.00062246810152)))
REPRESENTATION_ITEM('')
SURFACE()
);
#3726=(
BOUNDED_SURFACE()
B_SPLINE_SURFACE(3,2,((#249507,#249508,#249509),(#249510,#249511,#249512),
(#249513,#249514,#249515),(#249516,#249517,#249518),(#249519,#249520,#249521),
(#249522,#249523,#249524)),.UNSPECIFIED.,.F.,.F.,.F.)
B_SPLINE_SURFACE_WITH_KNOTS((4,2,4),(3,3),(-9.5138740635603E-18,0.000257652232350882,
0.000515304464701774),(0.,1.),.UNSPECIFIED.)
GEOMETRIC_REPRESENTATION_ITEM()
RATIONAL_B_SPLINE_SURFACE(((1.,0.874619707139393,1.),(1.,0.87486118043118,
1.),(1.,0.855455725920206,1.),(1.,0.794699358955927,1.),(1.,0.753768977788158,
1.),(1.,0.708712527163641,1.)))
REPRESENTATION_ITEM('')
SURFACE()
);
#3727=(
BOUNDED_SURFACE()
B_SPLINE_SURFACE(3,2,((#249530,#249531,#249532),(#249533,#249534,#249535),
(#249536,#249537,#249538),(#249539,#249540,#249541)),.UNSPECIFIED.,.F.,
 .F.,.F.)
B_SPLINE_SURFACE_WITH_KNOTS((4,4),(3,3),(0.,0.000397394373651898),(0.,1.),
 .UNSPECIFIED.)
GEOMETRIC_REPRESENTATION_ITEM()
RATIONAL_B_SPLINE_SURFACE(((1.,0.707106781186546,1.),(1.,0.707752587915892,
1.),(1.,0.708377654540671,1.),(1.,0.708689770883326,1.)))
REPRESENTATION_ITEM('')
SURFACE()
);
#3728=(
BOUNDED_SURFACE()
B_SPLINE_SURFACE(3,2,((#249543,#249544,#249545),(#249546,#249547,#249548),
(#249549,#249550,#249551),(#249552,#249553,#249554)),.UNSPECIFIED.,.F.,
 .F.,.F.)
B_SPLINE_SURFACE_WITH_KNOTS((4,4),(3,3),(0.,0.000511815456479774),(0.,1.00105873160096),
 .UNSPECIFIED.)
GEOMETRIC_REPRESENTATION_ITEM()
RATIONAL_B_SPLINE_SURFACE(((1.,0.70839452905603,1.0006174638542),(1.,0.708058564166566,
1.00061817524749),(1.,0.707430835371767,1.00061950444012),(1.,0.70679668588009,
1.00062084722833)))
REPRESENTATION_ITEM('')
SURFACE()
);
#3729=(
BOUNDED_SURFACE()
B_SPLINE_SURFACE(3,2,((#249560,#249561,#249562),(#249563,#249564,#249565),
(#249566,#249567,#249568),(#249569,#249570,#249571)),.UNSPECIFIED.,.F.,
 .F.,.F.)
B_SPLINE_SURFACE_WITH_KNOTS((4,4),(3,3),(0.,0.000397394465448298),(0.,1.),
 .UNSPECIFIED.)
GEOMETRIC_REPRESENTATION_ITEM()
RATIONAL_B_SPLINE_SURFACE(((1.,0.705498956110755,1.),(1.,0.705821764811781,
1.),(1.,0.706461952521135,1.),(1.,0.707106781186546,1.)))
REPRESENTATION_ITEM('')
SURFACE()
);
#3730=(
BOUNDED_SURFACE()
B_SPLINE_SURFACE(3,2,((#249577,#249578,#249579),(#249580,#249581,#249582),
(#249583,#249584,#249585),(#249586,#249587,#249588)),.UNSPECIFIED.,.F.,
 .F.,.F.)
B_SPLINE_SURFACE_WITH_KNOTS((4,4),(3,3),(-3.25260651745651E-18,0.000397394410828732),
(0.,1.),.UNSPECIFIED.)
GEOMETRIC_REPRESENTATION_ITEM()
RATIONAL_B_SPLINE_SURFACE(((1.,0.708689770883298,1.),(1.,0.708376440034509,
1.),(1.,0.707750498698393,1.),(1.,0.707106781186555,1.)))
REPRESENTATION_ITEM('')
SURFACE()
);
#3731=(
BOUNDED_SURFACE()
B_SPLINE_SURFACE(3,2,((#249594,#249595,#249596),(#249597,#249598,#249599),
(#249600,#249601,#249602),(#249603,#249604,#249605)),.UNSPECIFIED.,.F.,
 .F.,.F.)
B_SPLINE_SURFACE_WITH_KNOTS((4,4),(3,3),(0.,0.000511815090126188),(0.,1.00105592270402),
 .UNSPECIFIED.)
GEOMETRIC_REPRESENTATION_ITEM()
RATIONAL_B_SPLINE_SURFACE(((1.,0.705266242716956,1.00062243213192),(1.,
0.705584085908583,1.00062176089623),(1.,0.706182089449988,1.0006204980052),
(1.,0.706797508586943,1.00061919833512)))
REPRESENTATION_ITEM('')
SURFACE()
);
#3732=(
BOUNDED_SURFACE()
B_SPLINE_SURFACE(3,2,((#249607,#249608,#249609),(#249610,#249611,#249612),
(#249613,#249614,#249615),(#249616,#249617,#249618)),.UNSPECIFIED.,.F.,
 .F.,.F.)
B_SPLINE_SURFACE_WITH_KNOTS((4,4),(3,3),(0.,0.000397394428086639),(0.,1.),
 .UNSPECIFIED.)
GEOMETRIC_REPRESENTATION_ITEM()
RATIONAL_B_SPLINE_SURFACE(((1.,0.707106781186549,1.),(1.,0.706459846759092,
1.),(1.,0.705820510737292,1.),(1.,0.705498956110755,1.)))
REPRESENTATION_ITEM('')
SURFACE()
);
#3733=(
BOUNDED_SURFACE()
B_SPLINE_SURFACE(3,2,((#249624,#249625,#249626),(#249627,#249628,#249629),
(#249630,#249631,#249632),(#249633,#249634,#249635),(#249636,#249637,#249638),
(#249639,#249640,#249641)),.UNSPECIFIED.,.F.,.F.,.F.)
B_SPLINE_SURFACE_WITH_KNOTS((4,2,4),(3,3),(0.,0.000257953807872845,0.00051590761574569),
(0.,1.),.UNSPECIFIED.)
GEOMETRIC_REPRESENTATION_ITEM()
RATIONAL_B_SPLINE_SURFACE(((1.,0.874619707139393,1.),(1.,0.874834349679431,
1.),(1.,0.85468610415722,1.),(1.,0.792476597915739,1.),(1.,0.750887854594666,
1.),(1.,0.705585838031452,1.)))
REPRESENTATION_ITEM('')
SURFACE()
);
#3734=(
BOUNDED_SURFACE()
B_SPLINE_SURFACE(3,2,((#249647,#249648,#249649),(#249650,#249651,#249652),
(#249653,#249654,#249655),(#249656,#249657,#249658)),.UNSPECIFIED.,.F.,
 .F.,.F.)
B_SPLINE_SURFACE_WITH_KNOTS((4,4),(3,3),(0.,0.000511815437699155),(0.,1.00105881331839),
 .UNSPECIFIED.)
GEOMETRIC_REPRESENTATION_ITEM()
RATIONAL_B_SPLINE_SURFACE(((1.,0.706796661945596,1.00062089519866),(1.,
0.707430821224483,1.00061955228608),(1.,0.708058545829982,1.00061822299973),
(1.,0.708394505251979,1.00061751156311)))
REPRESENTATION_ITEM('')
SURFACE()
);
#3735=(
BOUNDED_SURFACE()
B_SPLINE_SURFACE(3,2,((#249660,#249661,#249662),(#249663,#249664,#249665),
(#249666,#249667,#249668),(#249669,#249670,#249671),(#249672,#249673,#249674),
(#249675,#249676,#249677)),.UNSPECIFIED.,.F.,.F.,.F.)
B_SPLINE_SURFACE_WITH_KNOTS((4,2,4),(3,3),(2.90024081139872E-18,0.00025691531753127,
0.000513830635062537),(0.,1.),.UNSPECIFIED.)
GEOMETRIC_REPRESENTATION_ITEM()
RATIONAL_B_SPLINE_SURFACE(((1.,0.70558583803146,1.),(1.,0.75090243354268,
1.),(1.,0.792329530082599,1.),(1.,0.854288401594135,1.),(1.,0.874998031125191,
1.),(1.,0.874619707139406,1.)))
REPRESENTATION_ITEM('')
SURFACE()
);
#3736=(
BOUNDED_SURFACE()
B_SPLINE_SURFACE(3,2,((#249683,#249684,#249685),(#249686,#249687,#249688),
(#249689,#249690,#249691),(#249692,#249693,#249694),(#249695,#249696,#249697),
(#249698,#249699,#249700)),.UNSPECIFIED.,.F.,.F.,.F.)
B_SPLINE_SURFACE_WITH_KNOTS((4,2,4),(3,3),(-3.95733792957209E-18,0.000256592814262151,
0.000513185628524305),(0.,1.),.UNSPECIFIED.)
GEOMETRIC_REPRESENTATION_ITEM()
RATIONAL_B_SPLINE_SURFACE(((1.,0.708712527163649,1.),(1.,0.753780902613286,
1.),(1.,0.794538995769611,1.),(1.,0.855070770330693,1.),(1.,0.87501842744564,
1.),(1.,0.874619707139394,1.)))
REPRESENTATION_ITEM('')
SURFACE()
);
#3737=(
BOUNDED_SURFACE()
B_SPLINE_SURFACE(3,2,((#249702,#249703,#249704),(#249705,#249706,#249707),
(#249708,#249709,#249710),(#249711,#249712,#249713)),.UNSPECIFIED.,.F.,
 .F.,.F.)
B_SPLINE_SURFACE_WITH_KNOTS((4,4),(3,3),(2.71050543121376E-20,0.000511815072430399),
(0.,1.00105598365803),.UNSPECIFIED.)
GEOMETRIC_REPRESENTATION_ITEM()
RATIONAL_B_SPLINE_SURFACE(((1.,0.706797490733933,1.00061923411655),(1.,
0.70618206214684,1.00062053388162),(1.,0.705584062769212,1.00062179683676),
(1.,0.705266224770693,1.00062246810022)))
REPRESENTATION_ITEM('')
SURFACE()
);
#3738=(
BOUNDED_SURFACE()
B_SPLINE_SURFACE(3,2,((#249719,#249720,#249721),(#249722,#249723,#249724),
(#249725,#249726,#249727),(#249728,#249729,#249730),(#249731,#249732,#249733),
(#249734,#249735,#249736)),.UNSPECIFIED.,.F.,.F.,.F.)
B_SPLINE_SURFACE_WITH_KNOTS((4,2,4),(3,3),(-3.21194893598831E-18,0.000257652232350884,
0.000515304464701772),(0.,1.),.UNSPECIFIED.)
GEOMETRIC_REPRESENTATION_ITEM()
RATIONAL_B_SPLINE_SURFACE(((1.,0.874619707139385,1.),(1.,0.87486118043075,
1.),(1.,0.855455725920803,1.),(1.,0.794699358955335,1.),(1.,0.753768977788572,
1.),(1.,0.708712527163662,1.)))
REPRESENTATION_ITEM('')
SURFACE()
);
#3739=(
BOUNDED_SURFACE()
B_SPLINE_SURFACE(3,2,((#249742,#249743,#249744),(#249745,#249746,#249747),
(#249748,#249749,#249750),(#249751,#249752,#249753)),.UNSPECIFIED.,.F.,
 .F.,.F.)
B_SPLINE_SURFACE_WITH_KNOTS((4,4),(3,3),(5.96311194867027E-19,0.000397394373651915),
(0.,1.),.UNSPECIFIED.)
GEOMETRIC_REPRESENTATION_ITEM()
RATIONAL_B_SPLINE_SURFACE(((1.,0.707106781186546,1.),(1.,0.707752587915887,
1.),(1.,0.708377654540691,1.),(1.,0.708689770883333,1.)))
REPRESENTATION_ITEM('')
SURFACE()
);
#3740=(
BOUNDED_SURFACE()
B_SPLINE_SURFACE(3,2,((#249755,#249756,#249757),(#249758,#249759,#249760),
(#249761,#249762,#249763),(#249764,#249765,#249766)),.UNSPECIFIED.,.F.,
 .F.,.F.)
B_SPLINE_SURFACE_WITH_KNOTS((4,4),(3,3),(-1.59919820441612E-18,0.000511815456479778),
(0.,1.00105873160197),.UNSPECIFIED.)
GEOMETRIC_REPRESENTATION_ITEM()
RATIONAL_B_SPLINE_SURFACE(((1.,0.708394529055743,1.00061746385479),(1.,
0.708058564166312,1.00061817524808),(1.,0.707430835371452,1.00061950444071),
(1.,0.706796685879791,1.00062084722892)))
REPRESENTATION_ITEM('')
SURFACE()
);
#3741=(
BOUNDED_SURFACE()
B_SPLINE_SURFACE(3,2,((#249772,#249773,#249774),(#249775,#249776,#249777),
(#249778,#249779,#249780),(#249781,#249782,#249783)),.UNSPECIFIED.,.F.,
 .F.,.F.)
B_SPLINE_SURFACE_WITH_KNOTS((4,4),(3,3),(3.27971157176865E-18,0.000397394465448314),
(0.,1.),.UNSPECIFIED.)
GEOMETRIC_REPRESENTATION_ITEM()
RATIONAL_B_SPLINE_SURFACE(((1.,0.705498956110724,1.),(1.,0.705821764811811,
1.),(1.,0.706461952521113,1.),(1.,0.70710678118654,1.)))
REPRESENTATION_ITEM('')
SURFACE()
);
#3742=(
BOUNDED_SURFACE()
B_SPLINE_SURFACE(3,2,((#249789,#249790,#249791),(#249792,#249793,#249794),
(#249795,#249796,#249797),(#249798,#249799,#249800)),.UNSPECIFIED.,.F.,
 .F.,.F.)
B_SPLINE_SURFACE_WITH_KNOTS((4,4),(3,3),(0.,0.000397394410828754),(0.,1.),
 .UNSPECIFIED.)
GEOMETRIC_REPRESENTATION_ITEM()
RATIONAL_B_SPLINE_SURFACE(((1.,0.708689770883333,1.),(1.,0.708376440034482,
1.),(1.,0.707750498698425,1.),(1.,0.707106781186548,1.)))
REPRESENTATION_ITEM('')
SURFACE()
);
#3743=(
BOUNDED_SURFACE()
B_SPLINE_SURFACE(3,2,((#249806,#249807,#249808),(#249809,#249810,#249811),
(#249812,#249813,#249814),(#249815,#249816,#249817)),.UNSPECIFIED.,.F.,
 .F.,.F.)
B_SPLINE_SURFACE_WITH_KNOTS((4,4),(3,3),(0.,0.000511815090126182),(0.,1.00105592270073),
 .UNSPECIFIED.)
GEOMETRIC_REPRESENTATION_ITEM()
RATIONAL_B_SPLINE_SURFACE(((1.,0.705266242717918,1.00062243212997),(1.,
0.705584085909569,1.00062176089429),(1.,0.706182089450925,1.00062049800326),
(1.,0.706797508587914,1.00061919833318)))
REPRESENTATION_ITEM('')
SURFACE()
);
#3744=(
BOUNDED_SURFACE()
B_SPLINE_SURFACE(3,2,((#249819,#249820,#249821),(#249822,#249823,#249824),
(#249825,#249826,#249827),(#249828,#249829,#249830)),.UNSPECIFIED.,.F.,
 .F.,.F.)
B_SPLINE_SURFACE_WITH_KNOTS((4,4),(3,3),(-7.26415455565288E-18,0.000397394428086632),
(0.,1.),.UNSPECIFIED.)
GEOMETRIC_REPRESENTATION_ITEM()
RATIONAL_B_SPLINE_SURFACE(((1.,0.707106781186548,1.),(1.,0.706459846759083,
1.),(1.,0.705820510737279,1.),(1.,0.705498956110751,1.)))
REPRESENTATION_ITEM('')
SURFACE()
);
#3745=(
BOUNDED_SURFACE()
B_SPLINE_SURFACE(3,2,((#249836,#249837,#249838),(#249839,#249840,#249841),
(#249842,#249843,#249844),(#249845,#249846,#249847),(#249848,#249849,#249850),
(#249851,#249852,#249853)),.UNSPECIFIED.,.F.,.F.,.F.)
B_SPLINE_SURFACE_WITH_KNOTS((4,2,4),(3,3),(0.,0.00025795380787284,0.00051590761574568),
(0.,1.),.UNSPECIFIED.)
GEOMETRIC_REPRESENTATION_ITEM()
RATIONAL_B_SPLINE_SURFACE(((1.,0.874619707139393,1.),(1.,0.874834349678958,
1.),(1.,0.854686104157849,1.),(1.,0.792476597915072,1.),(1.,0.750887854595184,
1.),(1.,0.705585838031448,1.)))
REPRESENTATION_ITEM('')
SURFACE()
);
#3746=(
BOUNDED_SURFACE()
B_SPLINE_SURFACE(3,2,((#249859,#249860,#249861),(#249862,#249863,#249864),
(#249865,#249866,#249867),(#249868,#249869,#249870)),.UNSPECIFIED.,.F.,
 .F.,.F.)
B_SPLINE_SURFACE_WITH_KNOTS((4,4),(3,3),(5.96311194867027E-19,0.000511815437699145),
(0.,1.00105881331926),.UNSPECIFIED.)
GEOMETRIC_REPRESENTATION_ITEM()
RATIONAL_B_SPLINE_SURFACE(((1.,0.706796661945347,1.00062089519917),(1.,
0.707430821224218,1.00061955228658),(1.,0.708058545829726,1.00061822300024),
(1.,0.708394505251735,1.00061751156362)))
REPRESENTATION_ITEM('')
SURFACE()
);
#3747=(
BOUNDED_SURFACE()
B_SPLINE_SURFACE(3,2,((#249872,#249873,#249874),(#249875,#249876,#249877),
(#249878,#249879,#249880),(#249881,#249882,#249883),(#249884,#249885,#249886),
(#249887,#249888,#249889)),.UNSPECIFIED.,.F.,.F.,.F.)
B_SPLINE_SURFACE_WITH_KNOTS((4,2,4),(3,3),(0.,0.000256915317531259,0.000513830635062518),
(0.,1.),.UNSPECIFIED.)
GEOMETRIC_REPRESENTATION_ITEM()
RATIONAL_B_SPLINE_SURFACE(((1.,0.705585838031445,1.),(1.,0.750902433542064,
1.),(1.,0.792329530083464,1.),(1.,0.854288401593278,1.),(1.,0.874998031125833,
1.),(1.,0.874619707139395,1.)))
REPRESENTATION_ITEM('')
SURFACE()
);
#3748=(
BOUNDED_SURFACE()
B_SPLINE_SURFACE(3,2,((#249895,#249896,#249897),(#249898,#249899,#249900),
(#249901,#249902,#249903),(#249904,#249905,#249906),(#249907,#249908,#249909),
(#249910,#249911,#249912)),.UNSPECIFIED.,.F.,.F.,.F.)
B_SPLINE_SURFACE_WITH_KNOTS((4,2,4),(3,3),(-3.52365706057789E-19,0.000256592814262156,
0.000513185628524312),(0.,1.),.UNSPECIFIED.)
GEOMETRIC_REPRESENTATION_ITEM()
RATIONAL_B_SPLINE_SURFACE(((1.,0.708712527163661,1.),(1.,0.753780902613628,
1.),(1.,0.794538995769124,1.),(1.,0.85507077033118,1.),(1.,0.875018427445262,
1.),(1.,0.874619707139395,1.)))
REPRESENTATION_ITEM('')
SURFACE()
);
#3749=(
BOUNDED_SURFACE()
B_SPLINE_SURFACE(3,2,((#249914,#249915,#249916),(#249917,#249918,#249919),
(#249920,#249921,#249922),(#249923,#249924,#249925)),.UNSPECIFIED.,.F.,
 .F.,.F.)
B_SPLINE_SURFACE_WITH_KNOTS((4,4),(3,3),(-5.42101086242752E-19,0.000511815072430401),
(0.,1.00105598365713),.UNSPECIFIED.)
GEOMETRIC_REPRESENTATION_ITEM()
RATIONAL_B_SPLINE_SURFACE(((1.,0.706797490734198,1.00061923411603),(1.,
0.706182062147102,1.00062053388109),(1.,0.705584062769515,1.00062179683623),
(1.,0.705266224770947,1.00062246809969)))
REPRESENTATION_ITEM('')
SURFACE()
);
#3750=(
BOUNDED_SURFACE()
B_SPLINE_SURFACE(3,2,((#249931,#249932,#249933),(#249934,#249935,#249936),
(#249937,#249938,#249939),(#249940,#249941,#249942),(#249943,#249944,#249945),
(#249946,#249947,#249948)),.UNSPECIFIED.,.F.,.F.,.F.)
B_SPLINE_SURFACE_WITH_KNOTS((4,2,4),(3,3),(-1.35525271560688E-20,0.00025765223235088,
0.00051530446470176),(0.,1.),.UNSPECIFIED.)
GEOMETRIC_REPRESENTATION_ITEM()
RATIONAL_B_SPLINE_SURFACE(((1.,0.874619707139398,1.),(1.,0.874861180431335,
1.),(1.,0.855455725920025,1.),(1.,0.794699358956114,1.),(1.,0.753768977787991,
1.),(1.,0.708712527163669,1.)))
REPRESENTATION_ITEM('')
SURFACE()
);
#3751=(
BOUNDED_SURFACE()
B_SPLINE_SURFACE(3,2,((#249954,#249955,#249956),(#249957,#249958,#249959),
(#249960,#249961,#249962),(#249963,#249964,#249965)),.UNSPECIFIED.,.F.,
 .F.,.F.)
B_SPLINE_SURFACE_WITH_KNOTS((4,4),(3,3),(0.,0.000397394373651909),(0.,1.),
 .UNSPECIFIED.)
GEOMETRIC_REPRESENTATION_ITEM()
RATIONAL_B_SPLINE_SURFACE(((1.,0.707106781186548,1.),(1.,0.707752587915889,
1.),(1.,0.708377654540692,1.),(1.,0.708689770883327,1.)))
REPRESENTATION_ITEM('')
SURFACE()
);
#3752=(
BOUNDED_SURFACE()
B_SPLINE_SURFACE(3,2,((#249967,#249968,#249969),(#249970,#249971,#249972),
(#249973,#249974,#249975),(#249976,#249977,#249978)),.UNSPECIFIED.,.F.,
 .F.,.F.)
B_SPLINE_SURFACE_WITH_KNOTS((4,4),(3,3),(0.,0.000511815456479789),(0.,1.00105873159976),
 .UNSPECIFIED.)
GEOMETRIC_REPRESENTATION_ITEM()
RATIONAL_B_SPLINE_SURFACE(((1.,0.708394529056382,1.0006174638535),(1.,0.708058564166943,
1.00061817524679),(1.,0.707430835372111,1.00061950443941),(1.,0.706796685880434,
1.00062084722763)))
REPRESENTATION_ITEM('')
SURFACE()
);
#3753=(
BOUNDED_SURFACE()
B_SPLINE_SURFACE(3,2,((#249984,#249985,#249986),(#249987,#249988,#249989),
(#249990,#249991,#249992),(#249993,#249994,#249995)),.UNSPECIFIED.,.F.,
 .F.,.F.)
B_SPLINE_SURFACE_WITH_KNOTS((4,4),(3,3),(0.,0.000397394465448301),(0.,1.),
 .UNSPECIFIED.)
GEOMETRIC_REPRESENTATION_ITEM()
RATIONAL_B_SPLINE_SURFACE(((1.,0.705498956110754,1.),(1.,0.705821764811775,
1.),(1.,0.706461952521147,1.),(1.,0.707106781186548,1.)))
REPRESENTATION_ITEM('')
SURFACE()
);
#3754=(
BOUNDED_SURFACE()
B_SPLINE_SURFACE(3,2,((#250001,#250002,#250003),(#250004,#250005,#250006),
(#250007,#250008,#250009),(#250010,#250011,#250012)),.UNSPECIFIED.,.F.,
 .F.,.F.)
B_SPLINE_SURFACE_WITH_KNOTS((4,4),(3,3),(0.,0.000397394410828734),(0.,1.),
 .UNSPECIFIED.)
GEOMETRIC_REPRESENTATION_ITEM()
RATIONAL_B_SPLINE_SURFACE(((1.,0.708689770883327,1.),(1.,0.708376440034502,
1.),(1.,0.707750498698397,1.),(1.,0.707106781186547,1.)))
REPRESENTATION_ITEM('')
SURFACE()
);
#3755=(
BOUNDED_SURFACE()
B_SPLINE_SURFACE(3,2,((#250018,#250019,#250020),(#250021,#250022,#250023),
(#250024,#250025,#250026),(#250027,#250028,#250029)),.UNSPECIFIED.,.F.,
 .F.,.F.)
B_SPLINE_SURFACE_WITH_KNOTS((4,4),(3,3),(0.,0.000511815090126177),(0.,1.00105592270346),
 .UNSPECIFIED.)
GEOMETRIC_REPRESENTATION_ITEM()
RATIONAL_B_SPLINE_SURFACE(((1.,0.705266242717117,1.00062243213158),(1.,
0.705584085908778,1.0006217608959),(1.,0.70618208945012,1.00062049800487),
(1.,0.706797508587112,1.00061919833479)))
REPRESENTATION_ITEM('')
SURFACE()
);
#3756=(
BOUNDED_SURFACE()
B_SPLINE_SURFACE(3,2,((#250031,#250032,#250033),(#250034,#250035,#250036),
(#250037,#250038,#250039),(#250040,#250041,#250042)),.UNSPECIFIED.,.F.,
 .F.,.F.)
B_SPLINE_SURFACE_WITH_KNOTS((4,4),(3,3),(0.,0.000397394428086637),(0.,1.),
 .UNSPECIFIED.)
GEOMETRIC_REPRESENTATION_ITEM()
RATIONAL_B_SPLINE_SURFACE(((1.,0.707106781186545,1.),(1.,0.706459846759095,
1.),(1.,0.705820510737284,1.),(1.,0.705498956110773,1.)))
REPRESENTATION_ITEM('')
SURFACE()
);
#3757=(
BOUNDED_SURFACE()
B_SPLINE_SURFACE(3,2,((#250048,#250049,#250050),(#250051,#250052,#250053),
(#250054,#250055,#250056),(#250057,#250058,#250059),(#250060,#250061,#250062),
(#250063,#250064,#250065)),.UNSPECIFIED.,.F.,.F.,.F.)
B_SPLINE_SURFACE_WITH_KNOTS((4,2,4),(3,3),(-1.35525271560688E-18,0.000257953807872841,
0.000515907615745683),(0.,1.),.UNSPECIFIED.)
GEOMETRIC_REPRESENTATION_ITEM()
RATIONAL_B_SPLINE_SURFACE(((1.,0.874619707139388,1.),(1.,0.874834349678696,
1.),(1.,0.85468610415819,1.),(1.,0.792476597914758,1.),(1.,0.750887854595417,
1.),(1.,0.705585838031446,1.)))
REPRESENTATION_ITEM('')
SURFACE()
);
#3758=(
BOUNDED_SURFACE()
B_SPLINE_SURFACE(3,2,((#250071,#250072,#250073),(#250074,#250075,#250076),
(#250077,#250078,#250079),(#250080,#250081,#250082)),.UNSPECIFIED.,.F.,
 .F.,.F.)
B_SPLINE_SURFACE_WITH_KNOTS((4,4),(3,3),(5.6920614055489E-19,0.000511815437699149),
(0.,1.00105881331655),.UNSPECIFIED.)
GEOMETRIC_REPRESENTATION_ITEM()
RATIONAL_B_SPLINE_SURFACE(((1.,0.706796661946143,1.00062089519758),(1.,
0.707430821225016,1.000619552285),(1.,0.708058545830524,1.00061822299866),
(1.,0.708394505252519,1.00061751156204)))
REPRESENTATION_ITEM('')
SURFACE()
);
#3759=(
BOUNDED_SURFACE()
B_SPLINE_SURFACE(3,2,((#250084,#250085,#250086),(#250087,#250088,#250089),
(#250090,#250091,#250092),(#250093,#250094,#250095),(#250096,#250097,#250098),
(#250099,#250100,#250101)),.UNSPECIFIED.,.F.,.F.,.F.)
B_SPLINE_SURFACE_WITH_KNOTS((4,2,4),(3,3),(2.71050543121376E-20,0.00025691531753127,
0.00051383063506254),(0.,1.),.UNSPECIFIED.)
GEOMETRIC_REPRESENTATION_ITEM()
RATIONAL_B_SPLINE_SURFACE(((1.,0.705585838031444,1.),(1.,0.750902433542877,
1.),(1.,0.792329530082359,1.),(1.,0.854288401594373,1.),(1.,0.87499803112502,
1.),(1.,0.874619707139415,1.)))
REPRESENTATION_ITEM('')
SURFACE()
);
#3760=(
BOUNDED_SURFACE()
B_SPLINE_SURFACE(3,2,((#250107,#250108,#250109),(#250110,#250111,#250112),
(#250113,#250114,#250115),(#250116,#250117,#250118),(#250119,#250120,#250121),
(#250122,#250123,#250124)),.UNSPECIFIED.,.F.,.F.,.F.)
B_SPLINE_SURFACE_WITH_KNOTS((4,2,4),(3,3),(-1.00017650411788E-17,0.000256592814262149,
0.000513185628524308),(0.,1.),.UNSPECIFIED.)
GEOMETRIC_REPRESENTATION_ITEM()
RATIONAL_B_SPLINE_SURFACE(((1.,0.708712527163658,1.),(1.,0.753780902613446,
1.),(1.,0.794538995769375,1.),(1.,0.855070770330916,1.),(1.,0.875018427445467,
1.),(1.,0.874619707139404,1.)))
REPRESENTATION_ITEM('')
SURFACE()
);
#3761=(
BOUNDED_SURFACE()
B_SPLINE_SURFACE(3,2,((#250126,#250127,#250128),(#250129,#250130,#250131),
(#250132,#250133,#250134),(#250135,#250136,#250137)),.UNSPECIFIED.,.F.,
 .F.,.F.)
B_SPLINE_SURFACE_WITH_KNOTS((4,4),(3,3),(-5.96311194867027E-19,0.000511815072430398),
(0.,1.00105598365647),.UNSPECIFIED.)
GEOMETRIC_REPRESENTATION_ITEM()
RATIONAL_B_SPLINE_SURFACE(((1.,0.706797490734389,1.00061923411564),(1.,
0.706182062147284,1.0006205338807),(1.,0.705584062769693,1.00062179683584),
(1.,0.705266224771152,1.0006224680993)))
REPRESENTATION_ITEM('')
SURFACE()
);
#3762=(
BOUNDED_SURFACE()
B_SPLINE_SURFACE(3,2,((#250143,#250144,#250145),(#250146,#250147,#250148),
(#250149,#250150,#250151),(#250152,#250153,#250154),(#250155,#250156,#250157),
(#250158,#250159,#250160)),.UNSPECIFIED.,.F.,.F.,.F.)
B_SPLINE_SURFACE_WITH_KNOTS((4,2,4),(3,3),(-8.53809210832335E-19,0.000257652232350881,
0.000515304464701762),(0.,1.),.UNSPECIFIED.)
GEOMETRIC_REPRESENTATION_ITEM()
RATIONAL_B_SPLINE_SURFACE(((1.,0.874619707139382,1.),(1.,0.874861180431399,
1.),(1.,0.85545572591994,1.),(1.,0.794699358956173,1.),(1.,0.753768977787953,
1.),(1.,0.708712527163656,1.)))
REPRESENTATION_ITEM('')
SURFACE()
);
#3763=(
BOUNDED_SURFACE()
B_SPLINE_SURFACE(3,2,((#250166,#250167,#250168),(#250169,#250170,#250171),
(#250172,#250173,#250174),(#250175,#250176,#250177)),.UNSPECIFIED.,.F.,
 .F.,.F.)
B_SPLINE_SURFACE_WITH_KNOTS((4,4),(3,3),(0.,0.000397394373651905),(0.,1.),
 .UNSPECIFIED.)
GEOMETRIC_REPRESENTATION_ITEM()
RATIONAL_B_SPLINE_SURFACE(((1.,0.707106781186545,1.),(1.,0.707752587915898,
1.),(1.,0.708377654540682,1.),(1.,0.70868977088332,1.)))
REPRESENTATION_ITEM('')
SURFACE()
);
#3764=(
BOUNDED_SURFACE()
B_SPLINE_SURFACE(3,2,((#250179,#250180,#250181),(#250182,#250183,#250184),
(#250185,#250186,#250187),(#250188,#250189,#250190)),.UNSPECIFIED.,.F.,
 .F.,.F.)
B_SPLINE_SURFACE_WITH_KNOTS((4,4),(3,3),(0.,0.00051181545647979),(0.,1.00105873159952),
 .UNSPECIFIED.)
GEOMETRIC_REPRESENTATION_ITEM()
RATIONAL_B_SPLINE_SURFACE(((1.,0.708394529056458,1.00061746385336),(1.,
0.708058564167018,1.00061817524665),(1.,0.707430835372176,1.00061950443927),
(1.,0.706796685880504,1.00062084722749)))
REPRESENTATION_ITEM('')
SURFACE()
);
#3765=(
BOUNDED_SURFACE()
B_SPLINE_SURFACE(3,2,((#250196,#250197,#250198),(#250199,#250200,#250201),
(#250202,#250203,#250204),(#250205,#250206,#250207)),.UNSPECIFIED.,.F.,
 .F.,.F.)
B_SPLINE_SURFACE_WITH_KNOTS((4,4),(3,3),(-5.6920614055489E-18,0.000397394465448292),
(0.,1.),.UNSPECIFIED.)
GEOMETRIC_REPRESENTATION_ITEM()
RATIONAL_B_SPLINE_SURFACE(((1.,0.705498956110746,1.),(1.,0.70582176481177,
1.),(1.,0.706461952521135,1.),(1.,0.70710678118655,1.)))
REPRESENTATION_ITEM('')
SURFACE()
);
#3766=(
BOUNDED_SURFACE()
B_SPLINE_SURFACE(3,2,((#250213,#250214,#250215),(#250216,#250217,#250218),
(#250219,#250220,#250221),(#250222,#250223,#250224)),.UNSPECIFIED.,.F.,
 .F.,.F.)
B_SPLINE_SURFACE_WITH_KNOTS((4,4),(3,3),(0.,0.000397394410828736),(0.,1.),
 .UNSPECIFIED.)
GEOMETRIC_REPRESENTATION_ITEM()
RATIONAL_B_SPLINE_SURFACE(((1.,0.708689770883334,1.),(1.,0.708376440034502,
1.),(1.,0.707750498698403,1.),(1.,0.707106781186548,1.)))
REPRESENTATION_ITEM('')
SURFACE()
);
#3767=(
BOUNDED_SURFACE()
B_SPLINE_SURFACE(3,2,((#250230,#250231,#250232),(#250233,#250234,#250235),
(#250236,#250237,#250238),(#250239,#250240,#250241)),.UNSPECIFIED.,.F.,
 .F.,.F.)
B_SPLINE_SURFACE_WITH_KNOTS((4,4),(3,3),(0.,0.000511815090126177),(0.,1.00105592270128),
 .UNSPECIFIED.)
GEOMETRIC_REPRESENTATION_ITEM()
RATIONAL_B_SPLINE_SURFACE(((1.,0.70526624271777,1.00062243213029),(1.,0.705584085909375,
1.00062176089461),(1.,0.706182089450778,1.00062049800358),(1.,0.706797508587752,
1.00061919833351)))
REPRESENTATION_ITEM('')
SURFACE()
);
#3768=(
BOUNDED_SURFACE()
B_SPLINE_SURFACE(3,2,((#250243,#250244,#250245),(#250246,#250247,#250248),
(#250249,#250250,#250251),(#250252,#250253,#250254)),.UNSPECIFIED.,.F.,
 .F.,.F.)
B_SPLINE_SURFACE_WITH_KNOTS((4,4),(3,3),(0.,0.000397394428086634),(0.,1.),
 .UNSPECIFIED.)
GEOMETRIC_REPRESENTATION_ITEM()
RATIONAL_B_SPLINE_SURFACE(((1.,0.707106781186548,1.),(1.,0.706459846759077,
1.),(1.,0.705820510737296,1.),(1.,0.705498956110732,1.)))
REPRESENTATION_ITEM('')
SURFACE()
);
#3769=(
BOUNDED_SURFACE()
B_SPLINE_SURFACE(3,2,((#250260,#250261,#250262),(#250263,#250264,#250265),
(#250266,#250267,#250268),(#250269,#250270,#250271),(#250272,#250273,#250274),
(#250275,#250276,#250277)),.UNSPECIFIED.,.F.,.F.,.F.)
B_SPLINE_SURFACE_WITH_KNOTS((4,2,4),(3,3),(0.,0.000257953807872852,0.000515907615745705),
(0.,1.),.UNSPECIFIED.)
GEOMETRIC_REPRESENTATION_ITEM()
RATIONAL_B_SPLINE_SURFACE(((1.,0.874619707139393,1.),(1.,0.874834349679286,
1.),(1.,0.854686104157385,1.),(1.,0.792476597915547,1.),(1.,0.750887854594819,
1.),(1.,0.705585838031429,1.)))
REPRESENTATION_ITEM('')
SURFACE()
);
#3770=(
BOUNDED_SURFACE()
B_SPLINE_SURFACE(3,2,((#250280,#250281,#250282),(#250283,#250284,#250285),
(#250286,#250287,#250288),(#250289,#250290,#250291)),.UNSPECIFIED.,.F.,
 .F.,.F.)
B_SPLINE_SURFACE_WITH_KNOTS((4,4),(3,3),(0.,0.000511815437699153),(0.,1.00105881331696),
 .UNSPECIFIED.)
GEOMETRIC_REPRESENTATION_ITEM()
RATIONAL_B_SPLINE_SURFACE(((1.,0.706796661946019,1.00062089519782),(1.,
0.70743082122491,1.00061955228524),(1.,0.708058545830392,1.0006182229989),
(1.,0.708394505252405,1.00061751156228)))
REPRESENTATION_ITEM('')
SURFACE()
);
#3771=(
BOUNDED_SURFACE()
B_SPLINE_SURFACE(3,2,((#250293,#250294,#250295),(#250296,#250297,#250298),
(#250299,#250300,#250301),(#250302,#250303,#250304),(#250305,#250306,#250307),
(#250308,#250309,#250310)),.UNSPECIFIED.,.F.,.F.,.F.)
B_SPLINE_SURFACE_WITH_KNOTS((4,2,4),(3,3),(0.,0.000256915317531262,0.000513830635062524),
(0.,1.),.UNSPECIFIED.)
GEOMETRIC_REPRESENTATION_ITEM()
RATIONAL_B_SPLINE_SURFACE(((1.,0.705585838031438,1.),(1.,0.750902433542942,
1.),(1.,0.792329530082252,1.),(1.,0.854288401594462,1.),(1.,0.874998031124935,
1.),(1.,0.874619707139393,1.)))
REPRESENTATION_ITEM('')
SURFACE()
);
#3772=(
BOUNDED_SURFACE()
B_SPLINE_SURFACE(3,2,((#250316,#250317,#250318),(#250319,#250320,#250321),
(#250322,#250323,#250324),(#250325,#250326,#250327),(#250328,#250329,#250330),
(#250331,#250332,#250333)),.UNSPECIFIED.,.F.,.F.,.F.)
B_SPLINE_SURFACE_WITH_KNOTS((4,2,4),(3,3),(-1.0435445910173E-17,0.000256592814262151,
0.000513185628524312),(0.,1.),.UNSPECIFIED.)
GEOMETRIC_REPRESENTATION_ITEM()
RATIONAL_B_SPLINE_SURFACE(((1.,0.708712527163666,1.),(1.,0.753780902613587,
1.),(1.,0.794538995769213,1.),(1.,0.855070770331108,1.),(1.,0.87501842744534,
1.),(1.,0.874619707139389,1.)))
REPRESENTATION_ITEM('')
SURFACE()
);
#3773=(
BOUNDED_SURFACE()
B_SPLINE_SURFACE(3,2,((#250334,#250335,#250336),(#250337,#250338,#250339),
(#250340,#250341,#250342),(#250343,#250344,#250345)),.UNSPECIFIED.,.F.,
 .F.,.F.)
B_SPLINE_SURFACE_WITH_KNOTS((4,4),(3,3),(-5.96311194867027E-19,0.000511815072430392),
(0.,1.00105598365949),.UNSPECIFIED.)
GEOMETRIC_REPRESENTATION_ITEM()
RATIONAL_B_SPLINE_SURFACE(((1.,0.706797490733506,1.00061923411741),(1.,
0.706182062146417,1.00062053388248),(1.,0.705584062768799,1.00062179683762),
(1.,0.705266224770268,1.00062246810108)))
REPRESENTATION_ITEM('')
SURFACE()
);
#3774=(
BOUNDED_SURFACE()
B_SPLINE_SURFACE(3,2,((#250349,#250350,#250351),(#250352,#250353,#250354),
(#250355,#250356,#250357),(#250358,#250359,#250360),(#250361,#250362,#250363),
(#250364,#250365,#250366)),.UNSPECIFIED.,.F.,.F.,.F.)
B_SPLINE_SURFACE_WITH_KNOTS((4,2,4),(3,3),(-6.36968776335234E-19,0.000257652232350878,
0.000515304464701756),(0.,1.),.UNSPECIFIED.)
GEOMETRIC_REPRESENTATION_ITEM()
RATIONAL_B_SPLINE_SURFACE(((1.,0.874619707139395,1.),(1.,0.874861180430727,
1.),(1.,0.855455725920841,1.),(1.,0.794699358955299,1.),(1.,0.753768977788615,
1.),(1.,0.708712527163659,1.)))
REPRESENTATION_ITEM('')
SURFACE()
);
#3775=(
BOUNDED_SURFACE()
B_SPLINE_SURFACE(3,2,((#250372,#250373,#250374),(#250375,#250376,#250377),
(#250378,#250379,#250380),(#250381,#250382,#250383)),.UNSPECIFIED.,.F.,
 .F.,.F.)
B_SPLINE_SURFACE_WITH_KNOTS((4,4),(3,3),(0.,0.000397394373651911),(0.,1.),
 .UNSPECIFIED.)
GEOMETRIC_REPRESENTATION_ITEM()
RATIONAL_B_SPLINE_SURFACE(((1.,0.707106781186548,1.),(1.,0.707752587915892,
1.),(1.,0.708377654540693,1.),(1.,0.708689770883328,1.)))
REPRESENTATION_ITEM('')
SURFACE()
);
#3776=(
BOUNDED_SURFACE()
B_SPLINE_SURFACE(3,2,((#250385,#250386,#250387),(#250388,#250389,#250390),
(#250391,#250392,#250393),(#250394,#250395,#250396)),.UNSPECIFIED.,.F.,
 .F.,.F.)
B_SPLINE_SURFACE_WITH_KNOTS((4,4),(3,3),(-5.61074624261249E-18,0.00051181545647978),
(0.,1.00105873160076),.UNSPECIFIED.)
GEOMETRIC_REPRESENTATION_ITEM()
RATIONAL_B_SPLINE_SURFACE(((1.,0.708394529056089,1.00061746385409),(1.,
0.70805856416664,1.00061817524738),(1.,0.70743083537182,1.00061950444),
(1.,0.70679668588014,1.00062084722821)))
REPRESENTATION_ITEM('')
SURFACE()
);
#3777=(
BOUNDED_SURFACE()
B_SPLINE_SURFACE(3,2,((#250402,#250403,#250404),(#250405,#250406,#250407),
(#250408,#250409,#250410),(#250411,#250412,#250413)),.UNSPECIFIED.,.F.,
 .F.,.F.)
B_SPLINE_SURFACE_WITH_KNOTS((4,4),(3,3),(-2.03287907341032E-18,0.000397394465448296),
(0.,1.),.UNSPECIFIED.)
GEOMETRIC_REPRESENTATION_ITEM()
RATIONAL_B_SPLINE_SURFACE(((1.,0.705498956110755,1.),(1.,0.70582176481177,
1.),(1.,0.706461952521151,1.),(1.,0.707106781186548,1.)))
REPRESENTATION_ITEM('')
SURFACE()
);
#3778=(
BOUNDED_SURFACE()
B_SPLINE_SURFACE(3,2,((#250419,#250420,#250421),(#250422,#250423,#250424),
(#250425,#250426,#250427),(#250428,#250429,#250430)),.UNSPECIFIED.,.F.,
 .F.,.F.)
B_SPLINE_SURFACE_WITH_KNOTS((4,4),(3,3),(0.,0.000397394410828736),(0.,1.),
 .UNSPECIFIED.)
GEOMETRIC_REPRESENTATION_ITEM()
RATIONAL_B_SPLINE_SURFACE(((1.,0.708689770883325,1.),(1.,0.708376440034479,
1.),(1.,0.707750498698413,1.),(1.,0.707106781186545,1.)))
REPRESENTATION_ITEM('')
SURFACE()
);
#3779=(
BOUNDED_SURFACE()
B_SPLINE_SURFACE(3,2,((#250436,#250437,#250438),(#250439,#250440,#250441),
(#250442,#250443,#250444),(#250445,#250446,#250447)),.UNSPECIFIED.,.F.,
 .F.,.F.)
B_SPLINE_SURFACE_WITH_KNOTS((4,4),(3,3),(0.,0.000511815090126176),(0.,1.00105592270094),
 .UNSPECIFIED.)
GEOMETRIC_REPRESENTATION_ITEM()
RATIONAL_B_SPLINE_SURFACE(((1.,0.705266242717862,1.00062243213009),(1.,
0.705584085909489,1.00062176089441),(1.,0.706182089450879,1.00062049800338),
(1.,0.706797508587852,1.00061919833331)))
REPRESENTATION_ITEM('')
SURFACE()
);
#3780=(
BOUNDED_SURFACE()
B_SPLINE_SURFACE(3,2,((#250449,#250450,#250451),(#250452,#250453,#250454),
(#250455,#250456,#250457),(#250458,#250459,#250460)),.UNSPECIFIED.,.F.,
 .F.,.F.)
B_SPLINE_SURFACE_WITH_KNOTS((4,4),(3,3),(-7.12862928409219E-18,0.000397394428086624),
(0.,1.),.UNSPECIFIED.)
GEOMETRIC_REPRESENTATION_ITEM()
RATIONAL_B_SPLINE_SURFACE(((1.,0.707106781186548,1.),(1.,0.7064598467591,
1.),(1.,0.705820510737274,1.),(1.,0.705498956110758,1.)))
REPRESENTATION_ITEM('')
SURFACE()
);
#3781=(
BOUNDED_SURFACE()
B_SPLINE_SURFACE(3,2,((#250466,#250467,#250468),(#250469,#250470,#250471),
(#250472,#250473,#250474),(#250475,#250476,#250477),(#250478,#250479,#250480),
(#250481,#250482,#250483)),.UNSPECIFIED.,.F.,.F.,.F.)
B_SPLINE_SURFACE_WITH_KNOTS((4,2,4),(3,3),(-8.53809210832335E-19,0.000257953807872848,
0.000515907615745697),(0.,1.),.UNSPECIFIED.)
GEOMETRIC_REPRESENTATION_ITEM()
RATIONAL_B_SPLINE_SURFACE(((1.,0.874619707139389,1.),(1.,0.874834349679475,
1.),(1.,0.854686104157152,1.),(1.,0.792476597915786,1.),(1.,0.750887854594648,
1.),(1.,0.705585838031442,1.)))
REPRESENTATION_ITEM('')
SURFACE()
);
#3782=(
BOUNDED_SURFACE()
B_SPLINE_SURFACE(3,2,((#250489,#250490,#250491),(#250492,#250493,#250494),
(#250495,#250496,#250497),(#250498,#250499,#250500)),.UNSPECIFIED.,.F.,
 .F.,.F.)
B_SPLINE_SURFACE_WITH_KNOTS((4,4),(3,3),(5.96311194867027E-19,0.00051181543769915),
(0.,1.00105881331694),.UNSPECIFIED.)
GEOMETRIC_REPRESENTATION_ITEM()
RATIONAL_B_SPLINE_SURFACE(((1.,0.70679666194603,1.0006208951978),(1.,0.707430821224897,
1.00061955228523),(1.,0.708058545830418,1.00061822299888),(1.,0.708394505252403,
1.00061751156226)))
REPRESENTATION_ITEM('')
SURFACE()
);
#3783=(
BOUNDED_SURFACE()
B_SPLINE_SURFACE(3,2,((#250502,#250503,#250504),(#250505,#250506,#250507),
(#250508,#250509,#250510),(#250511,#250512,#250513),(#250514,#250515,#250516),
(#250517,#250518,#250519)),.UNSPECIFIED.,.F.,.F.,.F.)
B_SPLINE_SURFACE_WITH_KNOTS((4,2,4),(3,3),(0.,0.000256915317531264,0.000513830635062528),
(0.,1.),.UNSPECIFIED.)
GEOMETRIC_REPRESENTATION_ITEM()
RATIONAL_B_SPLINE_SURFACE(((1.,0.705585838031432,1.),(1.,0.750902433542905,
1.),(1.,0.792329530082297,1.),(1.,0.854288401594434,1.),(1.,0.874998031124962,
1.),(1.,0.874619707139388,1.)))
REPRESENTATION_ITEM('')
SURFACE()
);
#3784=(
BOUNDED_SURFACE()
B_SPLINE_SURFACE(3,2,((#250525,#250526,#250527),(#250528,#250529,#250530),
(#250531,#250532,#250533),(#250534,#250535,#250536),(#250537,#250538,#250539),
(#250540,#250541,#250542)),.UNSPECIFIED.,.F.,.F.,.F.)
B_SPLINE_SURFACE_WITH_KNOTS((4,2,4),(3,3),(-2.62919026827735E-18,0.000256592814262154,
0.000513185628524311),(0.,1.),.UNSPECIFIED.)
GEOMETRIC_REPRESENTATION_ITEM()
RATIONAL_B_SPLINE_SURFACE(((1.,0.708712527163643,1.),(1.,0.753780902613486,
1.),(1.,0.79453899576934,1.),(1.,0.855070770330976,1.),(1.,0.875018427445422,
1.),(1.,0.874619707139395,1.)))
REPRESENTATION_ITEM('')
SURFACE()
);
#3785=(
BOUNDED_SURFACE()
B_SPLINE_SURFACE(3,2,((#250544,#250545,#250546),(#250547,#250548,#250549),
(#250550,#250551,#250552),(#250553,#250554,#250555)),.UNSPECIFIED.,.F.,
 .F.,.F.)
B_SPLINE_SURFACE_WITH_KNOTS((4,4),(3,3),(-5.42101086242752E-19,0.000511815072430395),
(0.,1.00105598365927),.UNSPECIFIED.)
GEOMETRIC_REPRESENTATION_ITEM()
RATIONAL_B_SPLINE_SURFACE(((1.,0.706797490733568,1.00061923411729),(1.,
0.706182062146479,1.00062053388235),(1.,0.705584062768855,1.00062179683749),
(1.,0.705266224770321,1.00062246810096)))
REPRESENTATION_ITEM('')
SURFACE()
);
#3786=(
BOUNDED_SURFACE()
B_SPLINE_SURFACE(3,2,((#250561,#250562,#250563),(#250564,#250565,#250566),
(#250567,#250568,#250569),(#250570,#250571,#250572),(#250573,#250574,#250575),
(#250576,#250577,#250578)),.UNSPECIFIED.,.F.,.F.,.F.)
B_SPLINE_SURFACE_WITH_KNOTS((4,2,4),(3,3),(1.35525271560688E-20,0.000257652232350878,
0.000515304464701755),(0.,1.),.UNSPECIFIED.)
GEOMETRIC_REPRESENTATION_ITEM()
RATIONAL_B_SPLINE_SURFACE(((1.,0.874619707139397,1.),(1.,0.874861180430768,
1.),(1.,0.855455725920795,1.),(1.,0.794699358955348,1.),(1.,0.753768977788566,
1.),(1.,0.708712527163672,1.)))
REPRESENTATION_ITEM('')
SURFACE()
);
#3787=(
BOUNDED_SURFACE()
B_SPLINE_SURFACE(3,2,((#250584,#250585,#250586),(#250587,#250588,#250589),
(#250590,#250591,#250592),(#250593,#250594,#250595)),.UNSPECIFIED.,.F.,
 .F.,.F.)
B_SPLINE_SURFACE_WITH_KNOTS((4,4),(3,3),(0.,0.000397394373651909),(0.,1.),
 .UNSPECIFIED.)
GEOMETRIC_REPRESENTATION_ITEM()
RATIONAL_B_SPLINE_SURFACE(((1.,0.707106781186548,1.),(1.,0.707752587915876,
1.),(1.,0.708377654540709,1.),(1.,0.708689770883337,1.)))
REPRESENTATION_ITEM('')
SURFACE()
);
#3788=(
BOUNDED_SURFACE()
B_SPLINE_SURFACE(3,2,((#250597,#250598,#250599),(#250600,#250601,#250602),
(#250603,#250604,#250605),(#250606,#250607,#250608)),.UNSPECIFIED.,.F.,
 .F.,.F.)
B_SPLINE_SURFACE_WITH_KNOTS((4,4),(3,3),(0.,0.000511815456479791),(0.,1.00105873160053),
 .UNSPECIFIED.)
GEOMETRIC_REPRESENTATION_ITEM()
RATIONAL_B_SPLINE_SURFACE(((1.,0.708394529056164,1.00061746385395),(1.,
0.708058564166729,1.00061817524724),(1.,0.707430835371884,1.00061950443987),
(1.,0.706796685880206,1.00062084722808)))
REPRESENTATION_ITEM('')
SURFACE()
);
#3789=(
BOUNDED_SURFACE()
B_SPLINE_SURFACE(3,2,((#250614,#250615,#250616),(#250617,#250618,#250619),
(#250620,#250621,#250622),(#250623,#250624,#250625)),.UNSPECIFIED.,.F.,
 .F.,.F.)
B_SPLINE_SURFACE_WITH_KNOTS((4,4),(3,3),(-7.72494047895922E-18,0.000397394465448296),
(0.,1.),.UNSPECIFIED.)
GEOMETRIC_REPRESENTATION_ITEM()
RATIONAL_B_SPLINE_SURFACE(((1.,0.705498956110744,1.),(1.,0.705821764811781,
1.),(1.,0.706461952521132,1.),(1.,0.707106781186548,1.)))
REPRESENTATION_ITEM('')
SURFACE()
);
#3790=(
BOUNDED_SURFACE()
B_SPLINE_SURFACE(3,2,((#250631,#250632,#250633),(#250634,#250635,#250636),
(#250637,#250638,#250639),(#250640,#250641,#250642)),.UNSPECIFIED.,.F.,
 .F.,.F.)
B_SPLINE_SURFACE_WITH_KNOTS((4,4),(3,3),(0.,0.000397394410828758),(0.,1.),
 .UNSPECIFIED.)
GEOMETRIC_REPRESENTATION_ITEM()
RATIONAL_B_SPLINE_SURFACE(((1.,0.708689770883337,1.),(1.,0.708376440034474,
1.),(1.,0.707750498698435,1.),(1.,0.707106781186543,1.)))
REPRESENTATION_ITEM('')
SURFACE()
);
#3791=(
BOUNDED_SURFACE()
B_SPLINE_SURFACE(3,2,((#250648,#250649,#250650),(#250651,#250652,#250653),
(#250654,#250655,#250656),(#250657,#250658,#250659)),.UNSPECIFIED.,.F.,
 .F.,.F.)
B_SPLINE_SURFACE_WITH_KNOTS((4,4),(3,3),(0.,0.000511815090126189),(0.,1.0010559227023),
 .UNSPECIFIED.)
GEOMETRIC_REPRESENTATION_ITEM()
RATIONAL_B_SPLINE_SURFACE(((1.,0.705266242717454,1.0006224321309),(1.,0.705584085909081,
1.00062176089521),(1.,0.706182089450486,1.00062049800418),(1.,0.706797508587448,
1.00061919833411)))
REPRESENTATION_ITEM('')
SURFACE()
);
#3792=(
BOUNDED_SURFACE()
B_SPLINE_SURFACE(3,2,((#250661,#250662,#250663),(#250664,#250665,#250666),
(#250667,#250668,#250669),(#250670,#250671,#250672)),.UNSPECIFIED.,.F.,
 .F.,.F.)
B_SPLINE_SURFACE_WITH_KNOTS((4,4),(3,3),(0.,0.000397394428086637),(0.,1.),
 .UNSPECIFIED.)
GEOMETRIC_REPRESENTATION_ITEM()
RATIONAL_B_SPLINE_SURFACE(((1.,0.707106781186548,1.),(1.,0.706459846759098,
1.),(1.,0.705820510737255,1.),(1.,0.705498956110766,1.)))
REPRESENTATION_ITEM('')
SURFACE()
);
#3793=(
BOUNDED_SURFACE()
B_SPLINE_SURFACE(3,2,((#250678,#250679,#250680),(#250681,#250682,#250683),
(#250684,#250685,#250686),(#250687,#250688,#250689),(#250690,#250691,#250692),
(#250693,#250694,#250695)),.UNSPECIFIED.,.F.,.F.,.F.)
B_SPLINE_SURFACE_WITH_KNOTS((4,2,4),(3,3),(0.,0.000257953807872852,0.000515907615745703),
(0.,1.),.UNSPECIFIED.)
GEOMETRIC_REPRESENTATION_ITEM()
RATIONAL_B_SPLINE_SURFACE(((1.,0.874619707139395,1.),(1.,0.874834349679212,
1.),(1.,0.854686104157491,1.),(1.,0.792476597915442,1.),(1.,0.750887854594872,
1.),(1.,0.705585838031449,1.)))
REPRESENTATION_ITEM('')
SURFACE()
);
#3794=(
BOUNDED_SURFACE()
B_SPLINE_SURFACE(3,2,((#250701,#250702,#250703),(#250704,#250705,#250706),
(#250707,#250708,#250709),(#250710,#250711,#250712)),.UNSPECIFIED.,.F.,
 .F.,.F.)
B_SPLINE_SURFACE_WITH_KNOTS((4,4),(3,3),(0.,0.00051181543769915),(0.,1.00105881331692),
 .UNSPECIFIED.)
GEOMETRIC_REPRESENTATION_ITEM()
RATIONAL_B_SPLINE_SURFACE(((1.,0.706796661946038,1.00062089519779),(1.,
0.707430821224895,1.00061955228521),(1.,0.708058545830441,1.00061822299887),
(1.,0.708394505252425,1.00061751156225)))
REPRESENTATION_ITEM('')
SURFACE()
);
#3795=(
BOUNDED_SURFACE()
B_SPLINE_SURFACE(3,2,((#250714,#250715,#250716),(#250717,#250718,#250719),
(#250720,#250721,#250722),(#250723,#250724,#250725),(#250726,#250727,#250728),
(#250729,#250730,#250731)),.UNSPECIFIED.,.F.,.F.,.F.)
B_SPLINE_SURFACE_WITH_KNOTS((4,2,4),(3,3),(0.,0.000256915317531259,0.000513830635062518),
(0.,1.),.UNSPECIFIED.)
GEOMETRIC_REPRESENTATION_ITEM()
RATIONAL_B_SPLINE_SURFACE(((1.,0.705585838031427,1.),(1.,0.750902433542276,
1.),(1.,0.792329530083153,1.),(1.,0.85428840159355,1.),(1.,0.874998031125595,
1.),(1.,0.874619707139398,1.)))
REPRESENTATION_ITEM('')
SURFACE()
);
#3796=(
BOUNDED_SURFACE()
B_SPLINE_SURFACE(3,2,((#250737,#250738,#250739),(#250740,#250741,#250742),
(#250743,#250744,#250745),(#250746,#250747,#250748),(#250749,#250750,#250751),
(#250752,#250753,#250754)),.UNSPECIFIED.,.F.,.F.,.F.)
B_SPLINE_SURFACE_WITH_KNOTS((4,2,4),(3,3),(0.,0.000256592814262156,0.000513185628524313),
(0.,1.),.UNSPECIFIED.)
GEOMETRIC_REPRESENTATION_ITEM()
RATIONAL_B_SPLINE_SURFACE(((1.,0.708712527163666,1.),(1.,0.753780902613626,
1.),(1.,0.794538995769145,1.),(1.,0.855070770331172,1.),(1.,0.875018427445286,
1.),(1.,0.874619707139399,1.)))
REPRESENTATION_ITEM('')
SURFACE()
);
#3797=(
BOUNDED_SURFACE()
B_SPLINE_SURFACE(3,2,((#250756,#250757,#250758),(#250759,#250760,#250761),
(#250762,#250763,#250764),(#250765,#250766,#250767)),.UNSPECIFIED.,.F.,
 .F.,.F.)
B_SPLINE_SURFACE_WITH_KNOTS((4,4),(3,3),(-5.42101086242752E-19,0.000511815072430406),
(0.,1.00105598365709),.UNSPECIFIED.)
GEOMETRIC_REPRESENTATION_ITEM()
RATIONAL_B_SPLINE_SURFACE(((1.,0.706797490734208,1.000619234116),(1.,0.706182062147114,
1.00062053388107),(1.,0.705584062769522,1.0006217968362),(1.,0.705266224770962,
1.00062246809967)))
REPRESENTATION_ITEM('')
SURFACE()
);
#3798=(
BOUNDED_SURFACE()
B_SPLINE_SURFACE(3,2,((#250773,#250774,#250775),(#250776,#250777,#250778),
(#250779,#250780,#250781),(#250782,#250783,#250784),(#250785,#250786,#250787),
(#250788,#250789,#250790)),.UNSPECIFIED.,.F.,.F.,.F.)
B_SPLINE_SURFACE_WITH_KNOTS((4,2,4),(3,3),(-1.77538105744501E-18,0.000257652232350876,
0.000515304464701753),(0.,1.),.UNSPECIFIED.)
GEOMETRIC_REPRESENTATION_ITEM()
RATIONAL_B_SPLINE_SURFACE(((1.,0.874619707139395,1.),(1.,0.874861180430488,
1.),(1.,0.85545572592118,1.),(1.,0.794699358954985,1.),(1.,0.753768977788849,
1.),(1.,0.708712527163682,1.)))
REPRESENTATION_ITEM('')
SURFACE()
);
#3799=(
BOUNDED_SURFACE()
B_SPLINE_SURFACE(3,2,((#250796,#250797,#250798),(#250799,#250800,#250801),
(#250802,#250803,#250804),(#250805,#250806,#250807)),.UNSPECIFIED.,.F.,
 .F.,.F.)
B_SPLINE_SURFACE_WITH_KNOTS((4,4),(3,3),(0.,0.000397394373651913),(0.,1.),
 .UNSPECIFIED.)
GEOMETRIC_REPRESENTATION_ITEM()
RATIONAL_B_SPLINE_SURFACE(((1.,0.707106781186552,1.),(1.,0.707752587915901,
1.),(1.,0.70837765454067,1.),(1.,0.708689770883329,1.)))
REPRESENTATION_ITEM('')
SURFACE()
);
#3800=(
BOUNDED_SURFACE()
B_SPLINE_SURFACE(3,2,((#250809,#250810,#250811),(#250812,#250813,#250814),
(#250815,#250816,#250817),(#250818,#250819,#250820)),.UNSPECIFIED.,.F.,
 .F.,.F.)
B_SPLINE_SURFACE_WITH_KNOTS((4,4),(3,3),(-5.20417042793042E-18,0.000511815456479787),
(0.,1.0010587315994),.UNSPECIFIED.)
GEOMETRIC_REPRESENTATION_ITEM()
RATIONAL_B_SPLINE_SURFACE(((1.,0.708394529056482,1.00061746385329),(1.,
0.708058564167038,1.00061817524658),(1.,0.707430835372215,1.0006195044392),
(1.,0.706796685880545,1.00062084722741)))
REPRESENTATION_ITEM('')
SURFACE()
);
#3801=(
BOUNDED_SURFACE()
B_SPLINE_SURFACE(3,2,((#250826,#250827,#250828),(#250829,#250830,#250831),
(#250832,#250833,#250834),(#250835,#250836,#250837)),.UNSPECIFIED.,.F.,
 .F.,.F.)
B_SPLINE_SURFACE_WITH_KNOTS((4,4),(3,3),(0.,0.00039739446544832),(0.,1.),
 .UNSPECIFIED.)
GEOMETRIC_REPRESENTATION_ITEM()
RATIONAL_B_SPLINE_SURFACE(((1.,0.705498956110773,1.),(1.,0.705821764811761,
1.),(1.,0.706461952521155,1.),(1.,0.707106781186548,1.)))
REPRESENTATION_ITEM('')
SURFACE()
);
#3802=(
BOUNDED_SURFACE()
B_SPLINE_SURFACE(3,2,((#250843,#250844,#250845),(#250846,#250847,#250848),
(#250849,#250850,#250851),(#250852,#250853,#250854)),.UNSPECIFIED.,.F.,
 .F.,.F.)
B_SPLINE_SURFACE_WITH_KNOTS((4,4),(3,3),(0.,0.000397394410828742),(0.,1.),
 .UNSPECIFIED.)
GEOMETRIC_REPRESENTATION_ITEM()
RATIONAL_B_SPLINE_SURFACE(((1.,0.708689770883327,1.),(1.,0.708376440034486,
1.),(1.,0.707750498698416,1.),(1.,0.70710678118654,1.)))
REPRESENTATION_ITEM('')
SURFACE()
);
#3803=(
BOUNDED_SURFACE()
B_SPLINE_SURFACE(3,2,((#250860,#250861,#250862),(#250863,#250864,#250865),
(#250866,#250867,#250868),(#250869,#250870,#250871)),.UNSPECIFIED.,.F.,
 .F.,.F.)
B_SPLINE_SURFACE_WITH_KNOTS((4,4),(3,3),(0.,0.000511815090126184),(0.,1.00105592270038),
 .UNSPECIFIED.)
GEOMETRIC_REPRESENTATION_ITEM()
RATIONAL_B_SPLINE_SURFACE(((1.,0.705266242718023,1.00062243212977),(1.,
0.705584085909628,1.00062176089409),(1.,0.706182089451054,1.00062049800306),
(1.,0.706797508588024,1.00061919833298)))
REPRESENTATION_ITEM('')
SURFACE()
);
#3804=(
BOUNDED_SURFACE()
B_SPLINE_SURFACE(3,2,((#250873,#250874,#250875),(#250876,#250877,#250878),
(#250879,#250880,#250881),(#250882,#250883,#250884)),.UNSPECIFIED.,.F.,
 .F.,.F.)
B_SPLINE_SURFACE_WITH_KNOTS((4,4),(3,3),(-5.96311194867027E-19,0.000397394428086628),
(0.,1.),.UNSPECIFIED.)
GEOMETRIC_REPRESENTATION_ITEM()
RATIONAL_B_SPLINE_SURFACE(((1.,0.70710678118654,1.),(1.,0.706459846759098,
1.),(1.,0.705820510737268,1.),(1.,0.705498956110756,1.)))
REPRESENTATION_ITEM('')
SURFACE()
);
#3805=(
BOUNDED_SURFACE()
B_SPLINE_SURFACE(3,2,((#250890,#250891,#250892),(#250893,#250894,#250895),
(#250896,#250897,#250898),(#250899,#250900,#250901),(#250902,#250903,#250904),
(#250905,#250906,#250907)),.UNSPECIFIED.,.F.,.F.,.F.)
B_SPLINE_SURFACE_WITH_KNOTS((4,2,4),(3,3),(0.,0.00025795380787285,0.000515907615745701),
(0.,1.),.UNSPECIFIED.)
GEOMETRIC_REPRESENTATION_ITEM()
RATIONAL_B_SPLINE_SURFACE(((1.,0.874619707139394,1.),(1.,0.874834349679145,
1.),(1.,0.854686104157602,1.),(1.,0.792476597915341,1.),(1.,0.750887854594964,
1.),(1.,0.705585838031464,1.)))
REPRESENTATION_ITEM('')
SURFACE()
);
#3806=(
BOUNDED_SURFACE()
B_SPLINE_SURFACE(3,2,((#250913,#250914,#250915),(#250916,#250917,#250918),
(#250919,#250920,#250921),(#250922,#250923,#250924)),.UNSPECIFIED.,.F.,
 .F.,.F.)
B_SPLINE_SURFACE_WITH_KNOTS((4,4),(3,3),(0.,0.000511815437699155),(0.,1.00105881331637),
 .UNSPECIFIED.)
GEOMETRIC_REPRESENTATION_ITEM()
RATIONAL_B_SPLINE_SURFACE(((1.,0.706796661946191,1.00062089519747),(1.,
0.707430821225076,1.00061955228489),(1.,0.708058545830567,1.00061822299855),
(1.,0.708394505252572,1.00061751156193)))
REPRESENTATION_ITEM('')
SURFACE()
);
#3807=(
BOUNDED_SURFACE()
B_SPLINE_SURFACE(3,2,((#250926,#250927,#250928),(#250929,#250930,#250931),
(#250932,#250933,#250934),(#250935,#250936,#250937),(#250938,#250939,#250940),
(#250941,#250942,#250943)),.UNSPECIFIED.,.F.,.F.,.F.)
B_SPLINE_SURFACE_WITH_KNOTS((4,2,4),(3,3),(2.71050543121376E-20,0.000256915317531261,
0.000513830635062521),(0.,1.),.UNSPECIFIED.)
GEOMETRIC_REPRESENTATION_ITEM()
RATIONAL_B_SPLINE_SURFACE(((1.,0.705585838031446,1.),(1.,0.750902433542993,
1.),(1.,0.792329530082176,1.),(1.,0.854288401594561,1.),(1.,0.87499803112487,
1.),(1.,0.874619707139384,1.)))
REPRESENTATION_ITEM('')
SURFACE()
);
#3808=(
BOUNDED_SURFACE()
B_SPLINE_SURFACE(3,2,((#250949,#250950,#250951),(#250952,#250953,#250954),
(#250955,#250956,#250957),(#250958,#250959,#250960),(#250961,#250962,#250963),
(#250964,#250965,#250966)),.UNSPECIFIED.,.F.,.F.,.F.)
B_SPLINE_SURFACE_WITH_KNOTS((4,2,4),(3,3),(-2.5207700510288E-18,0.000256592814262154,
0.000513185628524311),(0.,1.),.UNSPECIFIED.)
GEOMETRIC_REPRESENTATION_ITEM()
RATIONAL_B_SPLINE_SURFACE(((1.,0.708712527163663,1.),(1.,0.753780902613565,
1.),(1.,0.794538995769234,1.),(1.,0.85507077033108,1.),(1.,0.87501842744533,
1.),(1.,0.874619707139398,1.)))
REPRESENTATION_ITEM('')
SURFACE()
);
#3809=(
BOUNDED_SURFACE()
B_SPLINE_SURFACE(3,2,((#250968,#250969,#250970),(#250971,#250972,#250973),
(#250974,#250975,#250976),(#250977,#250978,#250979)),.UNSPECIFIED.,.F.,
 .F.,.F.)
B_SPLINE_SURFACE_WITH_KNOTS((4,4),(3,3),(-5.6920614055489E-19,0.000511815072430393),
(0.,1.00105598365897),.UNSPECIFIED.)
GEOMETRIC_REPRESENTATION_ITEM()
RATIONAL_B_SPLINE_SURFACE(((1.,0.706797490733658,1.00061923411711),(1.,
0.706182062146592,1.00062053388217),(1.,0.705584062768913,1.00062179683731),
(1.,0.705266224770416,1.00062246810078)))
REPRESENTATION_ITEM('')
SURFACE()
);
#3810=(
BOUNDED_SURFACE()
B_SPLINE_SURFACE(3,2,((#250985,#250986,#250987),(#250988,#250989,#250990),
(#250991,#250992,#250993),(#250994,#250995,#250996),(#250997,#250998,#250999),
(#251000,#251001,#251002)),.UNSPECIFIED.,.F.,.F.,.F.)
B_SPLINE_SURFACE_WITH_KNOTS((4,2,4),(3,3),(-3.41523684332934E-18,0.000257652232350878,
0.00051530446470176),(0.,1.),.UNSPECIFIED.)
GEOMETRIC_REPRESENTATION_ITEM()
RATIONAL_B_SPLINE_SURFACE(((1.,0.874619707139395,1.),(1.,0.874861180430739,
1.),(1.,0.855455725920833,1.),(1.,0.794699358955319,1.),(1.,0.753768977788611,
1.),(1.,0.708712527163663,1.)))
REPRESENTATION_ITEM('')
SURFACE()
);
#3811=(
BOUNDED_SURFACE()
B_SPLINE_SURFACE(3,2,((#251008,#251009,#251010),(#251011,#251012,#251013),
(#251014,#251015,#251016),(#251017,#251018,#251019)),.UNSPECIFIED.,.F.,
 .F.,.F.)
B_SPLINE_SURFACE_WITH_KNOTS((4,4),(3,3),(0.,0.000397394373651901),(0.,1.),
 .UNSPECIFIED.)
GEOMETRIC_REPRESENTATION_ITEM()
RATIONAL_B_SPLINE_SURFACE(((1.,0.707106781186549,1.),(1.,0.707752587915924,
1.),(1.,0.70837765454066,1.),(1.,0.708689770883335,1.)))
REPRESENTATION_ITEM('')
SURFACE()
);
#3812=(
BOUNDED_SURFACE()
B_SPLINE_SURFACE(3,2,((#251021,#251022,#251023),(#251024,#251025,#251026),
(#251027,#251028,#251029),(#251030,#251031,#251032)),.UNSPECIFIED.,.F.,
 .F.,.F.)
B_SPLINE_SURFACE_WITH_KNOTS((4,4),(3,3),(-5.61074624261249E-18,0.000511815456479779),
(0.,1.00105873160044),.UNSPECIFIED.)
GEOMETRIC_REPRESENTATION_ITEM()
RATIONAL_B_SPLINE_SURFACE(((1.,0.708394529056196,1.0006174638539),(1.,0.708058564166725,
1.00061817524719),(1.,0.707430835371925,1.00061950443981),(1.,0.706796685880237,
1.00062084722802)))
REPRESENTATION_ITEM('')
SURFACE()
);
#3813=(
BOUNDED_SURFACE()
B_SPLINE_SURFACE(3,2,((#251038,#251039,#251040),(#251041,#251042,#251043),
(#251044,#251045,#251046),(#251047,#251048,#251049)),.UNSPECIFIED.,.F.,
 .F.,.F.)
B_SPLINE_SURFACE_WITH_KNOTS((4,4),(3,3),(0.,0.000397394465448301),(0.,1.),
 .UNSPECIFIED.)
GEOMETRIC_REPRESENTATION_ITEM()
RATIONAL_B_SPLINE_SURFACE(((1.,0.705498956110749,1.),(1.,0.70582176481179,
1.),(1.,0.706461952521136,1.),(1.,0.707106781186549,1.)))
REPRESENTATION_ITEM('')
SURFACE()
);
#3814=(
BOUNDED_SURFACE()
B_SPLINE_SURFACE(3,2,((#251055,#251056,#251057),(#251058,#251059,#251060),
(#251061,#251062,#251063),(#251064,#251065,#251066)),.UNSPECIFIED.,.F.,
 .F.,.F.)
B_SPLINE_SURFACE_WITH_KNOTS((4,4),(3,3),(0.,0.000397394410828748),(0.,1.),
 .UNSPECIFIED.)
GEOMETRIC_REPRESENTATION_ITEM()
RATIONAL_B_SPLINE_SURFACE(((1.,0.708689770883332,1.),(1.,0.708376440034477,
1.),(1.,0.707750498698426,1.),(1.,0.707106781186546,1.)))
REPRESENTATION_ITEM('')
SURFACE()
);
#3815=(
BOUNDED_SURFACE()
B_SPLINE_SURFACE(3,2,((#251072,#251073,#251074),(#251075,#251076,#251077),
(#251078,#251079,#251080),(#251081,#251082,#251083)),.UNSPECIFIED.,.F.,
 .F.,.F.)
B_SPLINE_SURFACE_WITH_KNOTS((4,4),(3,3),(3.19839640883224E-18,0.00051181509012619),
(0.,1.00105592270332),.UNSPECIFIED.)
GEOMETRIC_REPRESENTATION_ITEM()
RATIONAL_B_SPLINE_SURFACE(((1.,0.705266242717177,1.0006224321315),(1.,0.705584085908736,
1.00062176089582),(1.,0.706182089450218,1.00062049800479),(1.,0.706797508587152,
1.00061919833471)))
REPRESENTATION_ITEM('')
SURFACE()
);
#3816=(
BOUNDED_SURFACE()
B_SPLINE_SURFACE(3,2,((#251085,#251086,#251087),(#251088,#251089,#251090),
(#251091,#251092,#251093),(#251094,#251095,#251096)),.UNSPECIFIED.,.F.,
 .F.,.F.)
B_SPLINE_SURFACE_WITH_KNOTS((4,4),(3,3),(0.,0.000397394428086631),(0.,1.),
 .UNSPECIFIED.)
GEOMETRIC_REPRESENTATION_ITEM()
RATIONAL_B_SPLINE_SURFACE(((1.,0.707106781186546,1.),(1.,0.706459846759087,
1.),(1.,0.705820510737286,1.),(1.,0.705498956110744,1.)))
REPRESENTATION_ITEM('')
SURFACE()
);
#3817=(
BOUNDED_SURFACE()
B_SPLINE_SURFACE(3,2,((#251102,#251103,#251104),(#251105,#251106,#251107),
(#251108,#251109,#251110),(#251111,#251112,#251113),(#251114,#251115,#251116),
(#251117,#251118,#251119)),.UNSPECIFIED.,.F.,.F.,.F.)
B_SPLINE_SURFACE_WITH_KNOTS((4,2,4),(3,3),(0.,0.000257953807872843,0.000515907615745686),
(0.,1.),.UNSPECIFIED.)
GEOMETRIC_REPRESENTATION_ITEM()
RATIONAL_B_SPLINE_SURFACE(((1.,0.874619707139386,1.),(1.,0.874834349679186,
1.),(1.,0.854686104157541,1.),(1.,0.792476597915398,1.),(1.,0.750887854594977,
1.),(1.,0.705585838031422,1.)))
REPRESENTATION_ITEM('')
SURFACE()
);
#3818=(
BOUNDED_SURFACE()
B_SPLINE_SURFACE(3,2,((#251125,#251126,#251127),(#251128,#251129,#251130),
(#251131,#251132,#251133),(#251134,#251135,#251136)),.UNSPECIFIED.,.F.,
 .F.,.F.)
B_SPLINE_SURFACE_WITH_KNOTS((4,4),(3,3),(5.6920614055489E-19,0.000511815437699156),
(0.,1.00105881331822),.UNSPECIFIED.)
GEOMETRIC_REPRESENTATION_ITEM()
RATIONAL_B_SPLINE_SURFACE(((1.,0.706796661945643,1.00062089519855),(1.,
0.707430821224538,1.00061955228597),(1.,0.708058545830045,1.00061822299963),
(1.,0.708394505252033,1.00061751156301)))
REPRESENTATION_ITEM('')
SURFACE()
);
#3819=(
BOUNDED_SURFACE()
B_SPLINE_SURFACE(3,2,((#251138,#251139,#251140),(#251141,#251142,#251143),
(#251144,#251145,#251146),(#251147,#251148,#251149),(#251150,#251151,#251152),
(#251153,#251154,#251155)),.UNSPECIFIED.,.F.,.F.,.F.)
B_SPLINE_SURFACE_WITH_KNOTS((4,2,4),(3,3),(2.71050543121376E-20,0.000256915317531261,
0.000513830635062521),(0.,1.),.UNSPECIFIED.)
GEOMETRIC_REPRESENTATION_ITEM()
RATIONAL_B_SPLINE_SURFACE(((1.,0.705585838031431,1.),(1.,0.750902433543086,
1.),(1.,0.792329530082085,1.),(1.,0.854288401594642,1.),(1.,0.874998031124819,
1.),(1.,0.874619707139387,1.)))
REPRESENTATION_ITEM('')
SURFACE()
);
#3820=(
BOUNDED_SURFACE()
B_SPLINE_SURFACE(3,2,((#251161,#251162,#251163),(#251164,#251165,#251166),
(#251167,#251168,#251169),(#251170,#251171,#251172),(#251173,#251174,#251175),
(#251176,#251177,#251178)),.UNSPECIFIED.,.F.,.F.,.F.)
B_SPLINE_SURFACE_WITH_KNOTS((4,2,4),(3,3),(-2.54787510534094E-18,0.000256592814262151,
0.000513185628524304),(0.,1.),.UNSPECIFIED.)
GEOMETRIC_REPRESENTATION_ITEM()
RATIONAL_B_SPLINE_SURFACE(((1.,0.70871252716367,1.),(1.,0.75378090261397,
1.),(1.,0.7945389957687,1.),(1.,0.855070770331624,1.),(1.,0.875018427444944,
1.),(1.,0.874619707139394,1.)))
REPRESENTATION_ITEM('')
SURFACE()
);
#3821=(
BOUNDED_SURFACE()
B_SPLINE_SURFACE(3,2,((#251180,#251181,#251182),(#251183,#251184,#251185),
(#251186,#251187,#251188),(#251189,#251190,#251191)),.UNSPECIFIED.,.F.,
 .F.,.F.)
B_SPLINE_SURFACE_WITH_KNOTS((4,4),(3,3),(-8.13151629364128E-20,0.000511815072430399),
(0.,1.00105598366107),.UNSPECIFIED.)
GEOMETRIC_REPRESENTATION_ITEM()
RATIONAL_B_SPLINE_SURFACE(((1.,0.706797490733043,1.00061923411834),(1.,
0.706182062145961,1.00062053388341),(1.,0.705584062768314,1.00062179683855),
(1.,0.705266224769801,1.00062246810202)))
REPRESENTATION_ITEM('')
SURFACE()
);
#3822=(
BOUNDED_SURFACE()
B_SPLINE_SURFACE(3,2,((#251197,#251198,#251199),(#251200,#251201,#251202),
(#251203,#251204,#251205),(#251206,#251207,#251208),(#251209,#251210,#251211),
(#251212,#251213,#251214)),.UNSPECIFIED.,.F.,.F.,.F.)
B_SPLINE_SURFACE_WITH_KNOTS((4,2,4),(3,3),(0.,0.000257652232350877,0.000515304464701754),
(0.,1.),.UNSPECIFIED.)
GEOMETRIC_REPRESENTATION_ITEM()
RATIONAL_B_SPLINE_SURFACE(((1.,0.874619707139387,1.),(1.,0.874861180430411,
1.),(1.,0.855455725921276,1.),(1.,0.794699358954857,1.),(1.,0.753768977788948,
1.),(1.,0.708712527163661,1.)))
REPRESENTATION_ITEM('')
SURFACE()
);
#3823=(
BOUNDED_SURFACE()
B_SPLINE_SURFACE(3,2,((#251220,#251221,#251222),(#251223,#251224,#251225),
(#251226,#251227,#251228),(#251229,#251230,#251231)),.UNSPECIFIED.,.F.,
 .F.,.F.)
B_SPLINE_SURFACE_WITH_KNOTS((4,4),(3,3),(5.96311194867027E-19,0.000397394373651902),
(0.,1.),.UNSPECIFIED.)
GEOMETRIC_REPRESENTATION_ITEM()
RATIONAL_B_SPLINE_SURFACE(((1.,0.707106781186558,1.),(1.,0.707752587915892,
1.),(1.,0.708377654540708,1.),(1.,0.708689770883314,1.)))
REPRESENTATION_ITEM('')
SURFACE()
);
#3824=(
BOUNDED_SURFACE()
B_SPLINE_SURFACE(3,2,((#251233,#251234,#251235),(#251236,#251237,#251238),
(#251239,#251240,#251241),(#251242,#251243,#251244)),.UNSPECIFIED.,.F.,
 .F.,.F.)
B_SPLINE_SURFACE_WITH_KNOTS((4,4),(3,3),(0.,0.000511815456479788),(0.,1.001058731602),
 .UNSPECIFIED.)
GEOMETRIC_REPRESENTATION_ITEM()
RATIONAL_B_SPLINE_SURFACE(((1.,0.708394529055739,1.00061746385481),(1.,
0.708058564166243,1.0006181752481),(1.,0.707430835371497,1.00061950444072),
(1.,0.706796685879771,1.00062084722894)))
REPRESENTATION_ITEM('')
SURFACE()
);
#3825=(
BOUNDED_SURFACE()
B_SPLINE_SURFACE(3,2,((#251250,#251251,#251252),(#251253,#251254,#251255),
(#251256,#251257,#251258),(#251259,#251260,#251261)),.UNSPECIFIED.,.F.,
 .F.,.F.)
B_SPLINE_SURFACE_WITH_KNOTS((4,4),(3,3),(-4.33680868994202E-19,0.000397394465448297),
(0.,1.),.UNSPECIFIED.)
GEOMETRIC_REPRESENTATION_ITEM()
RATIONAL_B_SPLINE_SURFACE(((1.,0.705498956110758,1.),(1.,0.705821764811795,
1.),(1.,0.706461952521142,1.),(1.,0.707106781186557,1.)))
REPRESENTATION_ITEM('')
SURFACE()
);
#3826=(
BOUNDED_SURFACE()
B_SPLINE_SURFACE(3,2,((#251267,#251268,#251269),(#251270,#251271,#251272),
(#251273,#251274,#251275),(#251276,#251277,#251278)),.UNSPECIFIED.,.F.,
 .F.,.F.)
B_SPLINE_SURFACE_WITH_KNOTS((4,4),(3,3),(0.,0.000397394410828731),(0.,1.),
 .UNSPECIFIED.)
GEOMETRIC_REPRESENTATION_ITEM()
RATIONAL_B_SPLINE_SURFACE(((1.,0.708689770883321,1.),(1.,0.708376440034491,
1.),(1.,0.707750498698422,1.),(1.,0.707106781186546,1.)))
REPRESENTATION_ITEM('')
SURFACE()
);
#3827=(
BOUNDED_SURFACE()
B_SPLINE_SURFACE(3,2,((#251284,#251285,#251286),(#251287,#251288,#251289),
(#251290,#251291,#251292),(#251293,#251294,#251295)),.UNSPECIFIED.,.F.,
 .F.,.F.)
B_SPLINE_SURFACE_WITH_KNOTS((4,4),(3,3),(1.19262238973405E-18,0.000511815090126183),
(0.,1.00105592270195),.UNSPECIFIED.)
GEOMETRIC_REPRESENTATION_ITEM()
RATIONAL_B_SPLINE_SURFACE(((1.,0.705266242717556,1.00062243213069),(1.,
0.705584085909223,1.00062176089501),(1.,0.706182089450549,1.00062049800398),
(1.,0.706797508587564,1.0006191983339)))
REPRESENTATION_ITEM('')
SURFACE()
);
#3828=(
BOUNDED_SURFACE()
B_SPLINE_SURFACE(3,2,((#251297,#251298,#251299),(#251300,#251301,#251302),
(#251303,#251304,#251305),(#251306,#251307,#251308)),.UNSPECIFIED.,.F.,
 .F.,.F.)
B_SPLINE_SURFACE_WITH_KNOTS((4,4),(3,3),(-1.57209315010398E-17,0.000397394428086616),
(0.,1.),.UNSPECIFIED.)
GEOMETRIC_REPRESENTATION_ITEM()
RATIONAL_B_SPLINE_SURFACE(((1.,0.707106781186557,1.),(1.,0.70645984675906,
1.),(1.,0.705820510737312,1.),(1.,0.705498956110748,1.)))
REPRESENTATION_ITEM('')
SURFACE()
);
#3829=(
BOUNDED_SURFACE()
B_SPLINE_SURFACE(3,2,((#251314,#251315,#251316),(#251317,#251318,#251319),
(#251320,#251321,#251322),(#251323,#251324,#251325),(#251326,#251327,#251328),
(#251329,#251330,#251331)),.UNSPECIFIED.,.F.,.F.,.F.)
B_SPLINE_SURFACE_WITH_KNOTS((4,2,4),(3,3),(0.,0.000257953807872847,0.000515907615745694),
(0.,1.),.UNSPECIFIED.)
GEOMETRIC_REPRESENTATION_ITEM()
RATIONAL_B_SPLINE_SURFACE(((1.,0.874619707139392,1.),(1.,0.874834349679668,
1.),(1.,0.854686104156887,1.),(1.,0.792476597916051,1.),(1.,0.750887854594419,
1.),(1.,0.705585838031433,1.)))
REPRESENTATION_ITEM('')
SURFACE()
);
#3830=(
BOUNDED_SURFACE()
B_SPLINE_SURFACE(3,2,((#251337,#251338,#251339),(#251340,#251341,#251342),
(#251343,#251344,#251345),(#251346,#251347,#251348)),.UNSPECIFIED.,.F.,
 .F.,.F.)
B_SPLINE_SURFACE_WITH_KNOTS((4,4),(3,3),(5.6920614055489E-19,0.000511815437699143),
(0.,1.00105881331806),.UNSPECIFIED.)
GEOMETRIC_REPRESENTATION_ITEM()
RATIONAL_B_SPLINE_SURFACE(((1.,0.706796661945705,1.00062089519846),(1.,
0.707430821224546,1.00061955228588),(1.,0.708058545830125,1.00061822299954),
(1.,0.708394505252067,1.00061751156292)))
REPRESENTATION_ITEM('')
SURFACE()
);
#3831=(
BOUNDED_SURFACE()
B_SPLINE_SURFACE(3,2,((#251350,#251351,#251352),(#251353,#251354,#251355),
(#251356,#251357,#251358),(#251359,#251360,#251361),(#251362,#251363,#251364),
(#251365,#251366,#251367)),.UNSPECIFIED.,.F.,.F.,.F.)
B_SPLINE_SURFACE_WITH_KNOTS((4,2,4),(3,3),(0.,0.000256915317531259,0.000513830635062519),
(0.,1.),.UNSPECIFIED.)
GEOMETRIC_REPRESENTATION_ITEM()
RATIONAL_B_SPLINE_SURFACE(((1.,0.705585838031461,1.),(1.,0.750902433542499,
1.),(1.,0.79232953008284,1.),(1.,0.854288401593916,1.),(1.,0.874998031125362,
1.),(1.,0.874619707139391,1.)))
REPRESENTATION_ITEM('')
SURFACE()
);
#3832=(
BOUNDED_SURFACE()
B_SPLINE_SURFACE(3,2,((#251373,#251374,#251375),(#251376,#251377,#251378),
(#251379,#251380,#251381),(#251382,#251383,#251384),(#251385,#251386,#251387),
(#251388,#251389,#251390)),.UNSPECIFIED.,.F.,.F.,.F.)
B_SPLINE_SURFACE_WITH_KNOTS((4,2,4),(3,3),(-3.52365706057789E-19,0.000256592814262155,
0.00051318562852431),(0.,1.),.UNSPECIFIED.)
GEOMETRIC_REPRESENTATION_ITEM()
RATIONAL_B_SPLINE_SURFACE(((1.,0.708712527163665,1.),(1.,0.753780902613458,
1.),(1.,0.794538995769382,1.),(1.,0.855070770330922,1.),(1.,0.875018427445469,
1.),(1.,0.874619707139403,1.)))
REPRESENTATION_ITEM('')
SURFACE()
);
#3833=(
BOUNDED_SURFACE()
B_SPLINE_SURFACE(3,2,((#251392,#251393,#251394),(#251395,#251396,#251397),
(#251398,#251399,#251400),(#251401,#251402,#251403)),.UNSPECIFIED.,.F.,
 .F.,.F.)
B_SPLINE_SURFACE_WITH_KNOTS((4,4),(3,3),(0.,0.000511815072430388),(0.,1.0010559836583),
 .UNSPECIFIED.)
GEOMETRIC_REPRESENTATION_ITEM()
RATIONAL_B_SPLINE_SURFACE(((1.,0.706797490733863,1.00061923411672),(1.,
0.706182062146757,1.00062053388178),(1.,0.705584062769147,1.00062179683692),
(1.,0.70526622477061,1.00062246810038)))
REPRESENTATION_ITEM('')
SURFACE()
);
#3834=(
BOUNDED_SURFACE()
B_SPLINE_SURFACE(3,2,((#251409,#251410,#251411),(#251412,#251413,#251414),
(#251415,#251416,#251417),(#251418,#251419,#251420),(#251421,#251422,#251423),
(#251424,#251425,#251426)),.UNSPECIFIED.,.F.,.F.,.F.)
B_SPLINE_SURFACE_WITH_KNOTS((4,2,4),(3,3),(0.,0.000257652232350886,0.000515304464701772),
(0.,1.),.UNSPECIFIED.)
GEOMETRIC_REPRESENTATION_ITEM()
RATIONAL_B_SPLINE_SURFACE(((1.,0.874619707139385,1.),(1.,0.874861180430413,
1.),(1.,0.855455725921248,1.),(1.,0.794699358954868,1.),(1.,0.753768977788925,
1.),(1.,0.708712527163669,1.)))
REPRESENTATION_ITEM('')
SURFACE()
);
#3835=(
BOUNDED_SURFACE()
B_SPLINE_SURFACE(3,2,((#251432,#251433,#251434),(#251435,#251436,#251437),
(#251438,#251439,#251440),(#251441,#251442,#251443)),.UNSPECIFIED.,.F.,
 .F.,.F.)
B_SPLINE_SURFACE_WITH_KNOTS((4,4),(3,3),(-1.5748036555352E-17,0.000397394373651903),
(0.,1.),.UNSPECIFIED.)
GEOMETRIC_REPRESENTATION_ITEM()
RATIONAL_B_SPLINE_SURFACE(((1.,0.70710678118655,1.),(1.,0.70775258791589,
1.),(1.,0.70837765454068,1.),(1.,0.708689770883327,1.)))
REPRESENTATION_ITEM('')
SURFACE()
);
#3836=(
BOUNDED_SURFACE()
B_SPLINE_SURFACE(3,2,((#251445,#251446,#251447),(#251448,#251449,#251450),
(#251451,#251452,#251453),(#251454,#251455,#251456)),.UNSPECIFIED.,.F.,
 .F.,.F.)
B_SPLINE_SURFACE_WITH_KNOTS((4,4),(3,3),(-3.79470760369927E-19,0.000511815456479784),
(0.,1.00105873159937),.UNSPECIFIED.)
GEOMETRIC_REPRESENTATION_ITEM()
RATIONAL_B_SPLINE_SURFACE(((1.,0.708394529056501,1.00061746385327),(1.,
0.708058564167041,1.00061817524656),(1.,0.707430835372212,1.00061950443918),
(1.,0.70679668588055,1.0006208472274)))
REPRESENTATION_ITEM('')
SURFACE()
);
#3837=(
BOUNDED_SURFACE()
B_SPLINE_SURFACE(3,2,((#251462,#251463,#251464),(#251465,#251466,#251467),
(#251468,#251469,#251470),(#251471,#251472,#251473)),.UNSPECIFIED.,.F.,
 .F.,.F.)
B_SPLINE_SURFACE_WITH_KNOTS((4,4),(3,3),(-1.21972744404619E-18,0.000397394465448303),
(0.,1.),.UNSPECIFIED.)
GEOMETRIC_REPRESENTATION_ITEM()
RATIONAL_B_SPLINE_SURFACE(((1.,0.705498956110749,1.),(1.,0.705821764811809,
1.),(1.,0.70646195252111,1.),(1.,0.707106781186557,1.)))
REPRESENTATION_ITEM('')
SURFACE()
);
#3838=(
BOUNDED_SURFACE()
B_SPLINE_SURFACE(3,2,((#251479,#251480,#251481),(#251482,#251483,#251484),
(#251485,#251486,#251487),(#251488,#251489,#251490)),.UNSPECIFIED.,.F.,
 .F.,.F.)
B_SPLINE_SURFACE_WITH_KNOTS((4,4),(3,3),(0.,0.00039739441082874),(0.,1.),
 .UNSPECIFIED.)
GEOMETRIC_REPRESENTATION_ITEM()
RATIONAL_B_SPLINE_SURFACE(((1.,0.708689770883337,1.),(1.,0.708376440034467,
1.),(1.,0.70775049869843,1.),(1.,0.707106781186535,1.)))
REPRESENTATION_ITEM('')
SURFACE()
);
#3839=(
BOUNDED_SURFACE()
B_SPLINE_SURFACE(3,2,((#251496,#251497,#251498),(#251499,#251500,#251501),
(#251502,#251503,#251504),(#251505,#251506,#251507)),.UNSPECIFIED.,.F.,
 .F.,.F.)
B_SPLINE_SURFACE_WITH_KNOTS((4,4),(3,3),(0.,0.00051181509012618),(0.,1.00105592270322),
 .UNSPECIFIED.)
GEOMETRIC_REPRESENTATION_ITEM()
RATIONAL_B_SPLINE_SURFACE(((1.,0.705266242717196,1.00062243213144),(1.,
0.705584085908844,1.00062176089576),(1.,0.706182089450187,1.00062049800472),
(1.,0.706797508587171,1.00061919833465)))
REPRESENTATION_ITEM('')
SURFACE()
);
#3840=(
BOUNDED_SURFACE()
B_SPLINE_SURFACE(3,2,((#251509,#251510,#251511),(#251512,#251513,#251514),
(#251515,#251516,#251517),(#251518,#251519,#251520)),.UNSPECIFIED.,.F.,
 .F.,.F.)
B_SPLINE_SURFACE_WITH_KNOTS((4,4),(3,3),(0.,0.000397394428086653),(0.,1.),
 .UNSPECIFIED.)
GEOMETRIC_REPRESENTATION_ITEM()
RATIONAL_B_SPLINE_SURFACE(((1.,0.707106781186551,1.),(1.,0.706459846759095,
1.),(1.,0.705820510737328,1.),(1.,0.705498956110736,1.)))
REPRESENTATION_ITEM('')
SURFACE()
);
#3841=(
BOUNDED_SURFACE()
B_SPLINE_SURFACE(3,2,((#251526,#251527,#251528),(#251529,#251530,#251531),
(#251532,#251533,#251534),(#251535,#251536,#251537),(#251538,#251539,#251540),
(#251541,#251542,#251543)),.UNSPECIFIED.,.F.,.F.,.F.)
B_SPLINE_SURFACE_WITH_KNOTS((4,2,4),(3,3),(-5.14996031930615E-19,0.000257953807872846,
0.000515907615745692),(0.,1.),.UNSPECIFIED.)
GEOMETRIC_REPRESENTATION_ITEM()
RATIONAL_B_SPLINE_SURFACE(((1.,0.874619707139391,1.),(1.,0.874834349679085,
1.),(1.,0.854686104157701,1.),(1.,0.79247659791524,1.),(1.,0.75088785459503,
1.),(1.,0.705585838031485,1.)))
REPRESENTATION_ITEM('')
SURFACE()
);
#3842=(
BOUNDED_SURFACE()
B_SPLINE_SURFACE(3,2,((#251549,#251550,#251551),(#251552,#251553,#251554),
(#251555,#251556,#251557),(#251558,#251559,#251560)),.UNSPECIFIED.,.F.,
 .F.,.F.)
B_SPLINE_SURFACE_WITH_KNOTS((4,4),(3,3),(0.,0.000511815437699156),(0.,1.00105881331948),
 .UNSPECIFIED.)
GEOMETRIC_REPRESENTATION_ITEM()
RATIONAL_B_SPLINE_SURFACE(((1.,0.706796661945281,1.0006208951993),(1.,0.707430821224171,
1.00061955228671),(1.,0.708058545829648,1.00061822300037),(1.,0.708394505251669,
1.00061751156375)))
REPRESENTATION_ITEM('')
SURFACE()
);
#3843=(
BOUNDED_SURFACE()
B_SPLINE_SURFACE(3,2,((#251562,#251563,#251564),(#251565,#251566,#251567),
(#251568,#251569,#251570),(#251571,#251572,#251573),(#251574,#251575,#251576),
(#251577,#251578,#251579)),.UNSPECIFIED.,.F.,.F.,.F.)
B_SPLINE_SURFACE_WITH_KNOTS((4,2,4),(3,3),(2.87313575708659E-18,0.000256915317531265,
0.000513830635062527),(0.,1.),.UNSPECIFIED.)
GEOMETRIC_REPRESENTATION_ITEM()
RATIONAL_B_SPLINE_SURFACE(((1.,0.705585838031446,1.),(1.,0.750902433542731,
1.),(1.,0.792329530082549,1.),(1.,0.85428840159417,1.),(1.,0.874998031125167,
1.),(1.,0.874619707139405,1.)))
REPRESENTATION_ITEM('')
SURFACE()
);
#3844=(
BOUNDED_SURFACE()
B_SPLINE_SURFACE(3,2,((#251585,#251586,#251587),(#251588,#251589,#251590),
(#251591,#251592,#251593),(#251594,#251595,#251596),(#251597,#251598,#251599),
(#251600,#251601,#251602)),.UNSPECIFIED.,.F.,.F.,.F.)
B_SPLINE_SURFACE_WITH_KNOTS((4,2,4),(3,3),(-1.08962318334793E-17,0.000256592814262147,
0.000513185628524304),(0.,1.),.UNSPECIFIED.)
GEOMETRIC_REPRESENTATION_ITEM()
RATIONAL_B_SPLINE_SURFACE(((1.,0.708712527163664,1.),(1.,0.753780902613837,
1.),(1.,0.794538995768865,1.),(1.,0.855070770331436,1.),(1.,0.875018427445072,
1.),(1.,0.874619707139397,1.)))
REPRESENTATION_ITEM('')
SURFACE()
);
#3845=(
BOUNDED_SURFACE()
B_SPLINE_SURFACE(3,2,((#251604,#251605,#251606),(#251607,#251608,#251609),
(#251610,#251611,#251612),(#251613,#251614,#251615)),.UNSPECIFIED.,.F.,
 .F.,.F.)
B_SPLINE_SURFACE_WITH_KNOTS((4,4),(3,3),(0.,0.000511815072430403),(0.,1.0010559836591),
 .UNSPECIFIED.)
GEOMETRIC_REPRESENTATION_ITEM()
RATIONAL_B_SPLINE_SURFACE(((1.,0.706797490733619,1.00061923411719),(1.,
0.706182062146509,1.00062053388225),(1.,0.70558406276892,1.00062179683739),
(1.,0.705266224770374,1.00062246810086)))
REPRESENTATION_ITEM('')
SURFACE()
);
#3846=(
BOUNDED_SURFACE()
B_SPLINE_SURFACE(3,2,((#251621,#251622,#251623),(#251624,#251625,#251626),
(#251627,#251628,#251629),(#251630,#251631,#251632),(#251633,#251634,#251635),
(#251636,#251637,#251638)),.UNSPECIFIED.,.F.,.F.,.F.)
B_SPLINE_SURFACE_WITH_KNOTS((4,2,4),(3,3),(0.,0.000257652232350878,0.000515304464701757),
(0.,1.),.UNSPECIFIED.)
GEOMETRIC_REPRESENTATION_ITEM()
RATIONAL_B_SPLINE_SURFACE(((1.,0.874619707139383,1.),(1.,0.874861180430538,
1.),(1.,0.855455725921087,1.),(1.,0.794699358955036,1.),(1.,0.753768977788808,
1.),(1.,0.708712527163679,1.)))
REPRESENTATION_ITEM('')
SURFACE()
);
#3847=(
BOUNDED_SURFACE()
B_SPLINE_SURFACE(3,2,((#251644,#251645,#251646),(#251647,#251648,#251649),
(#251650,#251651,#251652),(#251653,#251654,#251655)),.UNSPECIFIED.,.F.,
 .F.,.F.)
B_SPLINE_SURFACE_WITH_KNOTS((4,4),(3,3),(5.96311194867027E-19,0.000397394373651916),
(0.,1.),.UNSPECIFIED.)
GEOMETRIC_REPRESENTATION_ITEM()
RATIONAL_B_SPLINE_SURFACE(((1.,0.707106781186549,1.),(1.,0.70775258791589,
1.),(1.,0.708377654540699,1.),(1.,0.708689770883332,1.)))
REPRESENTATION_ITEM('')
SURFACE()
);
#3848=(
BOUNDED_SURFACE()
B_SPLINE_SURFACE(3,2,((#251657,#251658,#251659),(#251660,#251661,#251662),
(#251663,#251664,#251665),(#251666,#251667,#251668)),.UNSPECIFIED.,.F.,
 .F.,.F.)
B_SPLINE_SURFACE_WITH_KNOTS((4,4),(3,3),(-5.61074624261249E-18,0.000511815456479781),
(0.,1.00105873159944),.UNSPECIFIED.)
GEOMETRIC_REPRESENTATION_ITEM()
RATIONAL_B_SPLINE_SURFACE(((1.,0.708394529056449,1.00061746385331),(1.,
0.70805856416707,1.0006181752466),(1.,0.707430835372197,1.00061950443923),
(1.,0.706796685880541,1.00062084722744)))
REPRESENTATION_ITEM('')
SURFACE()
);
#3849=(
BOUNDED_SURFACE()
B_SPLINE_SURFACE(3,2,((#251674,#251675,#251676),(#251677,#251678,#251679),
(#251680,#251681,#251682),(#251683,#251684,#251685)),.UNSPECIFIED.,.F.,
 .F.,.F.)
B_SPLINE_SURFACE_WITH_KNOTS((4,4),(3,3),(0.,0.000397394465448315),(0.,1.),
 .UNSPECIFIED.)
GEOMETRIC_REPRESENTATION_ITEM()
RATIONAL_B_SPLINE_SURFACE(((1.,0.705498956110738,1.),(1.,0.7058217648118,
1.),(1.,0.706461952521122,1.),(1.,0.70710678118656,1.)))
REPRESENTATION_ITEM('')
SURFACE()
);
#3850=(
BOUNDED_SURFACE()
B_SPLINE_SURFACE(3,2,((#251691,#251692,#251693),(#251694,#251695,#251696),
(#251697,#251698,#251699),(#251700,#251701,#251702)),.UNSPECIFIED.,.F.,
 .F.,.F.)
B_SPLINE_SURFACE_WITH_KNOTS((4,4),(3,3),(0.,0.000397394410828751),(0.,1.),
 .UNSPECIFIED.)
GEOMETRIC_REPRESENTATION_ITEM()
RATIONAL_B_SPLINE_SURFACE(((1.,0.708689770883341,1.),(1.,0.708376440034478,
1.),(1.,0.707750498698437,1.),(1.,0.707106781186546,1.)))
REPRESENTATION_ITEM('')
SURFACE()
);
#3851=(
BOUNDED_SURFACE()
B_SPLINE_SURFACE(3,2,((#251708,#251709,#251710),(#251711,#251712,#251713),
(#251714,#251715,#251716),(#251717,#251718,#251719)),.UNSPECIFIED.,.F.,
 .F.,.F.)
B_SPLINE_SURFACE_WITH_KNOTS((4,4),(3,3),(-5.61074624261249E-18,0.000511815090126171),
(0.,1.00105592270005),.UNSPECIFIED.)
GEOMETRIC_REPRESENTATION_ITEM()
RATIONAL_B_SPLINE_SURFACE(((1.,0.705266242718099,1.00062243212957),(1.,
0.70558408590981,1.00062176089389),(1.,0.706182089451058,1.00062049800286),
(1.,0.706797508588123,1.00061919833279)))
REPRESENTATION_ITEM('')
SURFACE()
);
#3852=(
BOUNDED_SURFACE()
B_SPLINE_SURFACE(3,2,((#251721,#251722,#251723),(#251724,#251725,#251726),
(#251727,#251728,#251729),(#251730,#251731,#251732)),.UNSPECIFIED.,.F.,
 .F.,.F.)
B_SPLINE_SURFACE_WITH_KNOTS((4,4),(3,3),(-9.9475549325545E-18,0.000397394428086624),
(0.,1.),.UNSPECIFIED.)
GEOMETRIC_REPRESENTATION_ITEM()
RATIONAL_B_SPLINE_SURFACE(((1.,0.707106781186546,1.),(1.,0.706459846759125,
1.),(1.,0.705820510737227,1.),(1.,0.705498956110741,1.)))
REPRESENTATION_ITEM('')
SURFACE()
);
#3853=(
BOUNDED_SURFACE()
B_SPLINE_SURFACE(3,2,((#251738,#251739,#251740),(#251741,#251742,#251743),
(#251744,#251745,#251746),(#251747,#251748,#251749),(#251750,#251751,#251752),
(#251753,#251754,#251755)),.UNSPECIFIED.,.F.,.F.,.F.)
B_SPLINE_SURFACE_WITH_KNOTS((4,2,4),(3,3),(0.,0.000257953807872842,0.000515907615745685),
(0.,1.),.UNSPECIFIED.)
GEOMETRIC_REPRESENTATION_ITEM()
RATIONAL_B_SPLINE_SURFACE(((1.,0.87461970713939,1.),(1.,0.874834349679033,
1.),(1.,0.854686104157721,1.),(1.,0.792476597915213,1.),(1.,0.750887854595099,
1.),(1.,0.70558583803142,1.)))
REPRESENTATION_ITEM('')
SURFACE()
);
#3854=(
BOUNDED_SURFACE()
B_SPLINE_SURFACE(3,2,((#251761,#251762,#251763),(#251764,#251765,#251766),
(#251767,#251768,#251769),(#251770,#251771,#251772)),.UNSPECIFIED.,.F.,
 .F.,.F.)
B_SPLINE_SURFACE_WITH_KNOTS((4,4),(3,3),(0.,0.000511815437699156),(0.,1.0010588133186),
 .UNSPECIFIED.)
GEOMETRIC_REPRESENTATION_ITEM()
RATIONAL_B_SPLINE_SURFACE(((1.,0.70679666194554,1.00062089519878),(1.,0.707430821224428,
1.0006195522862),(1.,0.708058545829939,1.00061822299985),(1.,0.708394505251935,
1.00061751156323)))
REPRESENTATION_ITEM('')
SURFACE()
);
#3855=(
BOUNDED_SURFACE()
B_SPLINE_SURFACE(3,2,((#251774,#251775,#251776),(#251777,#251778,#251779),
(#251780,#251781,#251782),(#251783,#251784,#251785),(#251786,#251787,#251788),
(#251789,#251790,#251791)),.UNSPECIFIED.,.F.,.F.,.F.)
B_SPLINE_SURFACE_WITH_KNOTS((4,2,4),(3,3),(0.,0.000256915317531261,0.000513830635062522),
(0.,1.),.UNSPECIFIED.)
GEOMETRIC_REPRESENTATION_ITEM()
RATIONAL_B_SPLINE_SURFACE(((1.,0.705585838031441,1.),(1.,0.75090243354325,
1.),(1.,0.792329530081844,1.),(1.,0.854288401594898,1.),(1.,0.874998031124623,
1.),(1.,0.874619707139392,1.)))
REPRESENTATION_ITEM('')
SURFACE()
);
#3856=(
BOUNDED_SURFACE()
B_SPLINE_SURFACE(3,2,((#251797,#251798,#251799),(#251800,#251801,#251802),
(#251803,#251804,#251805),(#251806,#251807,#251808),(#251809,#251810,#251811),
(#251812,#251813,#251814)),.UNSPECIFIED.,.F.,.F.,.F.)
B_SPLINE_SURFACE_WITH_KNOTS((4,2,4),(3,3),(-1.00559751498031E-17,0.00025659281426215,
0.00051318562852431),(0.,1.),.UNSPECIFIED.)
GEOMETRIC_REPRESENTATION_ITEM()
RATIONAL_B_SPLINE_SURFACE(((1.,0.708712527163675,1.),(1.,0.753780902613865,
1.),(1.,0.79453899576883,1.),(1.,0.85507077033146,1.),(1.,0.875018427445065,
1.),(1.,0.874619707139397,1.)))
REPRESENTATION_ITEM('')
SURFACE()
);
#3857=(
BOUNDED_SURFACE()
B_SPLINE_SURFACE(3,2,((#251816,#251817,#251818),(#251819,#251820,#251821),
(#251822,#251823,#251824),(#251825,#251826,#251827)),.UNSPECIFIED.,.F.,
 .F.,.F.)
B_SPLINE_SURFACE_WITH_KNOTS((4,4),(3,3),(-5.23127548224256E-18,0.000511815072430389),
(0.,1.00105598365557),.UNSPECIFIED.)
GEOMETRIC_REPRESENTATION_ITEM()
RATIONAL_B_SPLINE_SURFACE(((1.,0.706797490734655,1.00061923411511),(1.,
0.706182062147555,1.00062053388017),(1.,0.705584062769966,1.00062179683531),
(1.,0.705266224771429,1.00062246809877)))
REPRESENTATION_ITEM('')
SURFACE()
);
#3858=(
BOUNDED_SURFACE()
B_SPLINE_SURFACE(3,2,((#251833,#251834,#251835),(#251836,#251837,#251838),
(#251839,#251840,#251841),(#251842,#251843,#251844),(#251845,#251846,#251847),
(#251848,#251849,#251850)),.UNSPECIFIED.,.F.,.F.,.F.)
B_SPLINE_SURFACE_WITH_KNOTS((4,2,4),(3,3),(0.,0.00025765223235088,0.00051530446470176),
(0.,1.),.UNSPECIFIED.)
GEOMETRIC_REPRESENTATION_ITEM()
RATIONAL_B_SPLINE_SURFACE(((1.,0.874619707139389,1.),(1.,0.874861180430388,
1.),(1.,0.8554557259213,1.),(1.,0.794699358954825,1.),(1.,0.753768977788989,
1.),(1.,0.708712527163643,1.)))
REPRESENTATION_ITEM('')
SURFACE()
);
#3859=(
BOUNDED_SURFACE()
B_SPLINE_SURFACE(3,2,((#251856,#251857,#251858),(#251859,#251860,#251861),
(#251862,#251863,#251864),(#251865,#251866,#251867)),.UNSPECIFIED.,.F.,
 .F.,.F.)
B_SPLINE_SURFACE_WITH_KNOTS((4,4),(3,3),(-1.46096242742422E-17,0.0003973943736519),
(0.,1.),.UNSPECIFIED.)
GEOMETRIC_REPRESENTATION_ITEM()
RATIONAL_B_SPLINE_SURFACE(((1.,0.707106781186549,1.),(1.,0.707752587915898,
1.),(1.,0.708377654540658,1.),(1.,0.708689770883325,1.)))
REPRESENTATION_ITEM('')
SURFACE()
);
#3860=(
BOUNDED_SURFACE()
B_SPLINE_SURFACE(3,2,((#251869,#251870,#251871),(#251872,#251873,#251874),
(#251875,#251876,#251877),(#251878,#251879,#251880)),.UNSPECIFIED.,.F.,
 .F.,.F.)
B_SPLINE_SURFACE_WITH_KNOTS((4,4),(3,3),(0.,0.000511815456479792),(0.,1.0010587315979),
 .UNSPECIFIED.)
GEOMETRIC_REPRESENTATION_ITEM()
RATIONAL_B_SPLINE_SURFACE(((1.,0.708394529056921,1.00061746385242),(1.,
0.708058564167515,1.00061817524571),(1.,0.7074308353726,1.00061950443833),
(1.,0.70679668588098,1.00062084722653)))
REPRESENTATION_ITEM('')
SURFACE()
);
#3861=(
BOUNDED_SURFACE()
B_SPLINE_SURFACE(3,2,((#251886,#251887,#251888),(#251889,#251890,#251891),
(#251892,#251893,#251894),(#251895,#251896,#251897)),.UNSPECIFIED.,.F.,
 .F.,.F.)
B_SPLINE_SURFACE_WITH_KNOTS((4,4),(3,3),(-4.06575814682064E-18,0.000397394465448297),
(0.,1.),.UNSPECIFIED.)
GEOMETRIC_REPRESENTATION_ITEM()
RATIONAL_B_SPLINE_SURFACE(((1.,0.705498956110766,1.),(1.,0.705821764811788,
1.),(1.,0.706461952521129,1.),(1.,0.707106781186549,1.)))
REPRESENTATION_ITEM('')
SURFACE()
);
#3862=(
BOUNDED_SURFACE()
B_SPLINE_SURFACE(3,2,((#251903,#251904,#251905),(#251906,#251907,#251908),
(#251909,#251910,#251911),(#251912,#251913,#251914)),.UNSPECIFIED.,.F.,
 .F.,.F.)
B_SPLINE_SURFACE_WITH_KNOTS((4,4),(3,3),(0.,0.000397394410828736),(0.,1.),
 .UNSPECIFIED.)
GEOMETRIC_REPRESENTATION_ITEM()
RATIONAL_B_SPLINE_SURFACE(((1.,0.708689770883297,1.),(1.,0.708376440034533,
1.),(1.,0.707750498698387,1.),(1.,0.707106781186545,1.)))
REPRESENTATION_ITEM('')
SURFACE()
);
#3863=(
BOUNDED_SURFACE()
B_SPLINE_SURFACE(3,2,((#251920,#251921,#251922),(#251923,#251924,#251925),
(#251926,#251927,#251928),(#251929,#251930,#251931)),.UNSPECIFIED.,.F.,
 .F.,.F.)
B_SPLINE_SURFACE_WITH_KNOTS((4,4),(3,3),(0.,0.000511815090126174),(0.,1.00105592270111),
 .UNSPECIFIED.)
GEOMETRIC_REPRESENTATION_ITEM()
RATIONAL_B_SPLINE_SURFACE(((1.,0.705266242717813,1.0006224321302),(1.,0.705584085909436,
1.00062176089451),(1.,0.706182089450826,1.00062049800348),(1.,0.706797508587798,
1.00061919833341)))
REPRESENTATION_ITEM('')
SURFACE()
);
#3864=(
BOUNDED_SURFACE()
B_SPLINE_SURFACE(3,2,((#251933,#251934,#251935),(#251936,#251937,#251938),
(#251939,#251940,#251941),(#251942,#251943,#251944)),.UNSPECIFIED.,.F.,
 .F.,.F.)
B_SPLINE_SURFACE_WITH_KNOTS((4,4),(3,3),(-1.05167610731094E-17,0.000397394428086628),
(0.,1.),.UNSPECIFIED.)
GEOMETRIC_REPRESENTATION_ITEM()
RATIONAL_B_SPLINE_SURFACE(((1.,0.707106781186545,1.),(1.,0.706459846759091,
1.),(1.,0.705820510737279,1.),(1.,0.705498956110751,1.)))
REPRESENTATION_ITEM('')
SURFACE()
);
#3865=(
BOUNDED_SURFACE()
B_SPLINE_SURFACE(3,2,((#251950,#251951,#251952),(#251953,#251954,#251955),
(#251956,#251957,#251958),(#251959,#251960,#251961),(#251962,#251963,#251964),
(#251965,#251966,#251967)),.UNSPECIFIED.,.F.,.F.,.F.)
B_SPLINE_SURFACE_WITH_KNOTS((4,2,4),(3,3),(0.,0.000257953807872849,0.000515907615745697),
(0.,1.),.UNSPECIFIED.)
GEOMETRIC_REPRESENTATION_ITEM()
RATIONAL_B_SPLINE_SURFACE(((1.,0.874619707139396,1.),(1.,0.874834349678808,
1.),(1.,0.854686104158024,1.),(1.,0.792476597914919,1.),(1.,0.750887854595303,
1.),(1.,0.705585838031442,1.)))
REPRESENTATION_ITEM('')
SURFACE()
);
#3866=(
BOUNDED_SURFACE()
B_SPLINE_SURFACE(3,2,((#251973,#251974,#251975),(#251976,#251977,#251978),
(#251979,#251980,#251981),(#251982,#251983,#251984)),.UNSPECIFIED.,.F.,
 .F.,.F.)
B_SPLINE_SURFACE_WITH_KNOTS((4,4),(3,3),(5.6920614055489E-19,0.000511815437699157),
(0.,1.00105881331715),.UNSPECIFIED.)
GEOMETRIC_REPRESENTATION_ITEM()
RATIONAL_B_SPLINE_SURFACE(((1.,0.706796661945948,1.00062089519793),(1.,
0.70743082122483,1.00061955228535),(1.,0.708058545830374,1.00061822299901),
(1.,0.708394505252341,1.00061751156239)))
REPRESENTATION_ITEM('')
SURFACE()
);
#3867=(
BOUNDED_SURFACE()
B_SPLINE_SURFACE(3,2,((#251986,#251987,#251988),(#251989,#251990,#251991),
(#251992,#251993,#251994),(#251995,#251996,#251997),(#251998,#251999,#252000),
(#252001,#252002,#252003)),.UNSPECIFIED.,.F.,.F.,.F.)
B_SPLINE_SURFACE_WITH_KNOTS((4,2,4),(3,3),(2.71050543121376E-20,0.000256915317531263,
0.000513830635062525),(0.,1.),.UNSPECIFIED.)
GEOMETRIC_REPRESENTATION_ITEM()
RATIONAL_B_SPLINE_SURFACE(((1.,0.705585838031425,1.),(1.,0.750902433542554,
1.),(1.,0.792329530082784,1.),(1.,0.854288401593908,1.),(1.,0.87499803112535,
1.),(1.,0.874619707139389,1.)))
REPRESENTATION_ITEM('')
SURFACE()
);
#3868=(
BOUNDED_SURFACE()
B_SPLINE_SURFACE(3,2,((#252009,#252010,#252011),(#252012,#252013,#252014),
(#252015,#252016,#252017),(#252018,#252019,#252020),(#252021,#252022,#252023),
(#252024,#252025,#252026)),.UNSPECIFIED.,.F.,.F.,.F.)
B_SPLINE_SURFACE_WITH_KNOTS((4,2,4),(3,3),(-2.16840434497101E-18,0.000256592814262163,
0.000513185628524328),(0.,1.),.UNSPECIFIED.)
GEOMETRIC_REPRESENTATION_ITEM()
RATIONAL_B_SPLINE_SURFACE(((1.,0.708712527163658,1.),(1.,0.753780902613584,
1.),(1.,0.794538995769163,1.),(1.,0.855070770331154,1.),(1.,0.875018427445297,
1.),(1.,0.874619707139398,1.)))
REPRESENTATION_ITEM('')
SURFACE()
);
#3869=(
BOUNDED_SURFACE()
B_SPLINE_SURFACE(3,2,((#252028,#252029,#252030),(#252031,#252032,#252033),
(#252034,#252035,#252036),(#252037,#252038,#252039)),.UNSPECIFIED.,.F.,
 .F.,.F.)
B_SPLINE_SURFACE_WITH_KNOTS((4,4),(3,3),(-5.80048162279745E-18,0.000511815072430405),
(0.,1.00105598365882),.UNSPECIFIED.)
GEOMETRIC_REPRESENTATION_ITEM()
RATIONAL_B_SPLINE_SURFACE(((1.,0.706797490733704,1.00061923411702),(1.,
0.706182062146584,1.00062053388208),(1.,0.705584062769038,1.00062179683722),
(1.,0.705266224770424,1.00062246810069)))
REPRESENTATION_ITEM('')
SURFACE()
);
#3870=(
BOUNDED_SURFACE()
B_SPLINE_SURFACE(3,2,((#252045,#252046,#252047),(#252048,#252049,#252050),
(#252051,#252052,#252053),(#252054,#252055,#252056),(#252057,#252058,#252059),
(#252060,#252061,#252062)),.UNSPECIFIED.,.F.,.F.,.F.)
B_SPLINE_SURFACE_WITH_KNOTS((4,2,4),(3,3),(1.35525271560688E-20,0.000257652232350883,
0.000515304464701766),(0.,1.),.UNSPECIFIED.)
GEOMETRIC_REPRESENTATION_ITEM()
RATIONAL_B_SPLINE_SURFACE(((1.,0.874619707139396,1.),(1.,0.874861180430779,
1.),(1.,0.855455725920777,1.),(1.,0.794699358955354,1.),(1.,0.753768977788557,
1.),(1.,0.708712527163675,1.)))
REPRESENTATION_ITEM('')
SURFACE()
);
#3871=(
BOUNDED_SURFACE()
B_SPLINE_SURFACE(3,2,((#252068,#252069,#252070),(#252071,#252072,#252073),
(#252074,#252075,#252076),(#252077,#252078,#252079)),.UNSPECIFIED.,.F.,
 .F.,.F.)
B_SPLINE_SURFACE_WITH_KNOTS((4,4),(3,3),(0.,0.000397394373651912),(0.,1.),
 .UNSPECIFIED.)
GEOMETRIC_REPRESENTATION_ITEM()
RATIONAL_B_SPLINE_SURFACE(((1.,0.707106781186537,1.),(1.,0.707752587915915,
1.),(1.,0.708377654540671,1.),(1.,0.708689770883328,1.)))
REPRESENTATION_ITEM('')
SURFACE()
);
#3872=(
BOUNDED_SURFACE()
B_SPLINE_SURFACE(3,2,((#252081,#252082,#252083),(#252084,#252085,#252086),
(#252087,#252088,#252089),(#252090,#252091,#252092)),.UNSPECIFIED.,.F.,
 .F.,.F.)
B_SPLINE_SURFACE_WITH_KNOTS((4,4),(3,3),(0.,0.000511815456479782),(0.,1.00105873159953),
 .UNSPECIFIED.)
GEOMETRIC_REPRESENTATION_ITEM()
RATIONAL_B_SPLINE_SURFACE(((1.,0.708394529056449,1.00061746385337),(1.,
0.708058564167009,1.00061817524665),(1.,0.707430835372194,1.00061950443928),
(1.,0.706796685880505,1.00062084722749)))
REPRESENTATION_ITEM('')
SURFACE()
);
#3873=(
BOUNDED_SURFACE()
B_SPLINE_SURFACE(3,2,((#252098,#252099,#252100),(#252101,#252102,#252103),
(#252104,#252105,#252106),(#252107,#252108,#252109)),.UNSPECIFIED.,.F.,
 .F.,.F.)
B_SPLINE_SURFACE_WITH_KNOTS((4,4),(3,3),(0.,0.000397394465448306),(0.,1.),
 .UNSPECIFIED.)
GEOMETRIC_REPRESENTATION_ITEM()
RATIONAL_B_SPLINE_SURFACE(((1.,0.705498956110769,1.),(1.,0.705821764811784,
1.),(1.,0.70646195252113,1.),(1.,0.70710678118655,1.)))
REPRESENTATION_ITEM('')
SURFACE()
);
#3874=(
BOUNDED_SURFACE()
B_SPLINE_SURFACE(3,2,((#252115,#252116,#252117),(#252118,#252119,#252120),
(#252121,#252122,#252123),(#252124,#252125,#252126)),.UNSPECIFIED.,.F.,
 .F.,.F.)
B_SPLINE_SURFACE_WITH_KNOTS((4,4),(3,3),(0.,0.000397394410828744),(0.,1.),
 .UNSPECIFIED.)
GEOMETRIC_REPRESENTATION_ITEM()
RATIONAL_B_SPLINE_SURFACE(((1.,0.708689770883331,1.),(1.,0.708376440034484,
1.),(1.,0.707750498698425,1.),(1.,0.707106781186545,1.)))
REPRESENTATION_ITEM('')
SURFACE()
);
#3875=(
BOUNDED_SURFACE()
B_SPLINE_SURFACE(3,2,((#252132,#252133,#252134),(#252135,#252136,#252137),
(#252138,#252139,#252140),(#252141,#252142,#252143)),.UNSPECIFIED.,.F.,
 .F.,.F.)
B_SPLINE_SURFACE_WITH_KNOTS((4,4),(3,3),(0.,0.000511815090126181),(0.,1.00105592270294),
 .UNSPECIFIED.)
GEOMETRIC_REPRESENTATION_ITEM()
RATIONAL_B_SPLINE_SURFACE(((1.,0.70526624271726,1.00062243213127),(1.,0.705584085908922,
1.00062176089559),(1.,0.706182089450262,1.00062049800456),(1.,0.706797508587264,
1.00061919833448)))
REPRESENTATION_ITEM('')
SURFACE()
);
#3876=(
BOUNDED_SURFACE()
B_SPLINE_SURFACE(3,2,((#252145,#252146,#252147),(#252148,#252149,#252150),
(#252151,#252152,#252153),(#252154,#252155,#252156)),.UNSPECIFIED.,.F.,
 .F.,.F.)
B_SPLINE_SURFACE_WITH_KNOTS((4,4),(3,3),(-6.50521303491303E-19,0.000397394428086628),
(0.,1.),.UNSPECIFIED.)
GEOMETRIC_REPRESENTATION_ITEM()
RATIONAL_B_SPLINE_SURFACE(((1.,0.707106781186545,1.),(1.,0.706459846759103,
1.),(1.,0.705820510737279,1.),(1.,0.705498956110742,1.)))
REPRESENTATION_ITEM('')
SURFACE()
);
#3877=(
BOUNDED_SURFACE()
B_SPLINE_SURFACE(3,2,((#252162,#252163,#252164),(#252165,#252166,#252167),
(#252168,#252169,#252170),(#252171,#252172,#252173),(#252174,#252175,#252176),
(#252177,#252178,#252179)),.UNSPECIFIED.,.F.,.F.,.F.)
B_SPLINE_SURFACE_WITH_KNOTS((4,2,4),(3,3),(-1.03947883287048E-17,0.000257953807872844,
0.000515907615745698),(0.,1.),.UNSPECIFIED.)
GEOMETRIC_REPRESENTATION_ITEM()
RATIONAL_B_SPLINE_SURFACE(((1.,0.874619707139394,1.),(1.,0.874834349678638,
1.),(1.,0.85468610415827,1.),(1.,0.792476597914672,1.),(1.,0.750887854595475,
1.),(1.,0.705585838031437,1.)))
REPRESENTATION_ITEM('')
SURFACE()
);
#3878=(
BOUNDED_SURFACE()
B_SPLINE_SURFACE(3,2,((#252185,#252186,#252187),(#252188,#252189,#252190),
(#252191,#252192,#252193),(#252194,#252195,#252196)),.UNSPECIFIED.,.F.,
 .F.,.F.)
B_SPLINE_SURFACE_WITH_KNOTS((4,4),(3,3),(0.,0.000511815437699158),(0.,1.00105881331704),
 .UNSPECIFIED.)
GEOMETRIC_REPRESENTATION_ITEM()
RATIONAL_B_SPLINE_SURFACE(((1.,0.706796661945995,1.00062089519786),(1.,
0.707430821224872,1.00061955228528),(1.,0.70805854583039,1.00061822299894),
(1.,0.708394505252366,1.00061751156232)))
REPRESENTATION_ITEM('')
SURFACE()
);
#3879=(
BOUNDED_SURFACE()
B_SPLINE_SURFACE(3,2,((#252198,#252199,#252200),(#252201,#252202,#252203),
(#252204,#252205,#252206),(#252207,#252208,#252209),(#252210,#252211,#252212),
(#252213,#252214,#252215)),.UNSPECIFIED.,.F.,.F.,.F.)
B_SPLINE_SURFACE_WITH_KNOTS((4,2,4),(3,3),(-1.43656787854329E-18,0.000256915317531251,
0.000513830635062504),(0.,1.),.UNSPECIFIED.)
GEOMETRIC_REPRESENTATION_ITEM()
RATIONAL_B_SPLINE_SURFACE(((1.,0.705585838031439,1.),(1.,0.750902433542744,
1.),(1.,0.792329530082503,1.),(1.,0.854288401594159,1.),(1.,0.874998031125173,
1.),(1.,0.874619707139391,1.)))
REPRESENTATION_ITEM('')
SURFACE()
);
#3880=(
BOUNDED_SURFACE()
B_SPLINE_SURFACE(3,2,((#252221,#252222,#252223),(#252224,#252225,#252226),
(#252227,#252228,#252229),(#252230,#252231,#252232),(#252233,#252234,#252235),
(#252236,#252237,#252238)),.UNSPECIFIED.,.F.,.F.,.F.)
B_SPLINE_SURFACE_WITH_KNOTS((4,2,4),(3,3),(-1.14654379740342E-17,0.000256592814262148,
0.000513185628524307),(0.,1.),.UNSPECIFIED.)
GEOMETRIC_REPRESENTATION_ITEM()
RATIONAL_B_SPLINE_SURFACE(((1.,0.708712527163693,1.),(1.,0.753780902613078,
1.),(1.,0.794538995769877,1.),(1.,0.855070770330416,1.),(1.,0.875018427445857,
1.),(1.,0.874619707139392,1.)))
REPRESENTATION_ITEM('')
SURFACE()
);
#3881=(
BOUNDED_SURFACE()
B_SPLINE_SURFACE(3,2,((#252240,#252241,#252242),(#252243,#252244,#252245),
(#252246,#252247,#252248),(#252249,#252250,#252251)),.UNSPECIFIED.,.F.,
 .F.,.F.)
B_SPLINE_SURFACE_WITH_KNOTS((4,4),(3,3),(-6.26126754610379E-18,0.000511815072430392),
(0.,1.00105598366083),.UNSPECIFIED.)
GEOMETRIC_REPRESENTATION_ITEM()
RATIONAL_B_SPLINE_SURFACE(((1.,0.706797490733103,1.0006192341182),(1.,0.706182062146034,
1.00062053388327),(1.,0.705584062768406,1.00062179683841),(1.,0.705266224769873,
1.00062246810188)))
REPRESENTATION_ITEM('')
SURFACE()
);
#3882=(
BOUNDED_SURFACE()
B_SPLINE_SURFACE(3,2,((#252257,#252258,#252259),(#252260,#252261,#252262),
(#252263,#252264,#252265),(#252266,#252267,#252268),(#252269,#252270,#252271),
(#252272,#252273,#252274)),.UNSPECIFIED.,.F.,.F.,.F.)
B_SPLINE_SURFACE_WITH_KNOTS((4,2,4),(3,3),(-5.42101086242752E-20,0.000257652232350875,
0.00051530446470175),(0.,1.),.UNSPECIFIED.)
GEOMETRIC_REPRESENTATION_ITEM()
RATIONAL_B_SPLINE_SURFACE(((1.,0.874619707139402,1.),(1.,0.874861180430557,
1.),(1.,0.855455725921085,1.),(1.,0.794699358955079,1.),(1.,0.753768977788781,
1.),(1.,0.708712527163674,1.)))
REPRESENTATION_ITEM('')
SURFACE()
);
#3883=(
BOUNDED_SURFACE()
B_SPLINE_SURFACE(3,2,((#252280,#252281,#252282),(#252283,#252284,#252285),
(#252286,#252287,#252288),(#252289,#252290,#252291)),.UNSPECIFIED.,.F.,
 .F.,.F.)
B_SPLINE_SURFACE_WITH_KNOTS((4,4),(3,3),(0.,0.000397394373651914),(0.,1.),
 .UNSPECIFIED.)
GEOMETRIC_REPRESENTATION_ITEM()
RATIONAL_B_SPLINE_SURFACE(((1.,0.70710678118655,1.),(1.,0.707752587915891,
1.),(1.,0.708377654540695,1.),(1.,0.708689770883321,1.)))
REPRESENTATION_ITEM('')
SURFACE()
);
#3884=(
BOUNDED_SURFACE()
B_SPLINE_SURFACE(3,2,((#252293,#252294,#252295),(#252296,#252297,#252298),
(#252299,#252300,#252301),(#252302,#252303,#252304)),.UNSPECIFIED.,.F.,
 .F.,.F.)
B_SPLINE_SURFACE_WITH_KNOTS((4,4),(3,3),(0.,0.000511815456479786),(0.,1.00105873160046),
 .UNSPECIFIED.)
GEOMETRIC_REPRESENTATION_ITEM()
RATIONAL_B_SPLINE_SURFACE(((1.,0.708394529056175,1.00061746385391),(1.,
0.708058564166742,1.0006181752472),(1.,0.707430835371885,1.00061950443983),
(1.,0.70679668588023,1.00062084722804)))
REPRESENTATION_ITEM('')
SURFACE()
);
#3885=(
BOUNDED_SURFACE()
B_SPLINE_SURFACE(3,2,((#252310,#252311,#252312),(#252313,#252314,#252315),
(#252316,#252317,#252318),(#252319,#252320,#252321)),.UNSPECIFIED.,.F.,
 .F.,.F.)
B_SPLINE_SURFACE_WITH_KNOTS((4,4),(3,3),(-7.31836466427715E-18,0.0003973944654483),
(0.,1.),.UNSPECIFIED.)
GEOMETRIC_REPRESENTATION_ITEM()
RATIONAL_B_SPLINE_SURFACE(((1.,0.705498956110778,1.),(1.,0.705821764811775,
1.),(1.,0.706461952521157,1.),(1.,0.70710678118655,1.)))
REPRESENTATION_ITEM('')
SURFACE()
);
#3886=(
BOUNDED_SURFACE()
B_SPLINE_SURFACE(3,2,((#252327,#252328,#252329),(#252330,#252331,#252332),
(#252333,#252334,#252335),(#252336,#252337,#252338)),.UNSPECIFIED.,.F.,
 .F.,.F.)
B_SPLINE_SURFACE_WITH_KNOTS((4,4),(3,3),(5.96311194867027E-19,0.000397394410828737),
(0.,1.),.UNSPECIFIED.)
GEOMETRIC_REPRESENTATION_ITEM()
RATIONAL_B_SPLINE_SURFACE(((1.,0.708689770883353,1.),(1.,0.70837644003448,
1.),(1.,0.707750498698424,1.),(1.,0.707106781186537,1.)))
REPRESENTATION_ITEM('')
SURFACE()
);
#3887=(
BOUNDED_SURFACE()
B_SPLINE_SURFACE(3,2,((#252344,#252345,#252346),(#252347,#252348,#252349),
(#252350,#252351,#252352),(#252353,#252354,#252355)),.UNSPECIFIED.,.F.,
 .F.,.F.)
B_SPLINE_SURFACE_WITH_KNOTS((4,4),(3,3),(0.,0.000511815090126187),(0.,1.00105592270198),
 .UNSPECIFIED.)
GEOMETRIC_REPRESENTATION_ITEM()
RATIONAL_B_SPLINE_SURFACE(((1.,0.705266242717543,1.00062243213071),(1.,
0.705584085909212,1.00062176089503),(1.,0.706182089450554,1.000620498004),
(1.,0.706797508587552,1.00061919833392)))
REPRESENTATION_ITEM('')
SURFACE()
);
#3888=(
BOUNDED_SURFACE()
B_SPLINE_SURFACE(3,2,((#252357,#252358,#252359),(#252360,#252361,#252362),
(#252363,#252364,#252365),(#252366,#252367,#252368)),.UNSPECIFIED.,.F.,
 .F.,.F.)
B_SPLINE_SURFACE_WITH_KNOTS((4,4),(3,3),(-1.75098650856409E-17,0.000397394428086613),
(0.,1.),.UNSPECIFIED.)
GEOMETRIC_REPRESENTATION_ITEM()
RATIONAL_B_SPLINE_SURFACE(((1.,0.707106781186552,1.),(1.,0.706459846759093,
1.),(1.,0.705820510737281,1.),(1.,0.705498956110746,1.)))
REPRESENTATION_ITEM('')
SURFACE()
);
#3889=(
BOUNDED_SURFACE()
B_SPLINE_SURFACE(3,2,((#252374,#252375,#252376),(#252377,#252378,#252379),
(#252380,#252381,#252382),(#252383,#252384,#252385),(#252386,#252387,#252388),
(#252389,#252390,#252391)),.UNSPECIFIED.,.F.,.F.,.F.)
B_SPLINE_SURFACE_WITH_KNOTS((4,2,4),(3,3),(0.,0.00025795380787285,0.0005159076157457),
(0.,1.),.UNSPECIFIED.)
GEOMETRIC_REPRESENTATION_ITEM()
RATIONAL_B_SPLINE_SURFACE(((1.,0.874619707139391,1.),(1.,0.874834349679644,
1.),(1.,0.854686104156943,1.),(1.,0.792476597916,1.),(1.,0.750887854594491,
1.),(1.,0.705585838031437,1.)))
REPRESENTATION_ITEM('')
SURFACE()
);
#3890=(
BOUNDED_SURFACE()
B_SPLINE_SURFACE(3,2,((#252397,#252398,#252399),(#252400,#252401,#252402),
(#252403,#252404,#252405),(#252406,#252407,#252408)),.UNSPECIFIED.,.F.,
 .F.,.F.)
B_SPLINE_SURFACE_WITH_KNOTS((4,4),(3,3),(0.,0.000511815437699156),(0.,1.00105881331732),
 .UNSPECIFIED.)
GEOMETRIC_REPRESENTATION_ITEM()
RATIONAL_B_SPLINE_SURFACE(((1.,0.706796661945905,1.00062089519803),(1.,
0.707430821224792,1.00061955228545),(1.,0.708058545830336,1.0006182229991),
(1.,0.708394505252305,1.00061751156248)))
REPRESENTATION_ITEM('')
SURFACE()
);
#3891=(
BOUNDED_SURFACE()
B_SPLINE_SURFACE(3,2,((#252410,#252411,#252412),(#252413,#252414,#252415),
(#252416,#252417,#252418),(#252419,#252420,#252421),(#252422,#252423,#252424),
(#252425,#252426,#252427)),.UNSPECIFIED.,.F.,.F.,.F.)
B_SPLINE_SURFACE_WITH_KNOTS((4,2,4),(3,3),(0.,0.000256915317531267,0.000513830635062535),
(0.,1.),.UNSPECIFIED.)
GEOMETRIC_REPRESENTATION_ITEM()
RATIONAL_B_SPLINE_SURFACE(((1.,0.70558583803144,1.),(1.,0.750902433541966,
1.),(1.,0.792329530083573,1.),(1.,0.854288401593169,1.),(1.,0.874998031125916,
1.),(1.,0.874619707139415,1.)))
REPRESENTATION_ITEM('')
SURFACE()
);
#3892=(
BOUNDED_SURFACE()
B_SPLINE_SURFACE(3,2,((#252433,#252434,#252435),(#252436,#252437,#252438),
(#252439,#252440,#252441),(#252442,#252443,#252444),(#252445,#252446,#252447),
(#252448,#252449,#252450)),.UNSPECIFIED.,.F.,.F.,.F.)
B_SPLINE_SURFACE_WITH_KNOTS((4,2,4),(3,3),(-4.68917439599981E-18,0.000256592814262156,
0.000513185628524317),(0.,1.),.UNSPECIFIED.)
GEOMETRIC_REPRESENTATION_ITEM()
RATIONAL_B_SPLINE_SURFACE(((1.,0.70871252716367,1.),(1.,0.753780902613218,
1.),(1.,0.794538995769711,1.),(1.,0.855070770330604,1.),(1.,0.87501842744571,
1.),(1.,0.874619707139392,1.)))
REPRESENTATION_ITEM('')
SURFACE()
);
#3893=(
BOUNDED_SURFACE()
B_SPLINE_SURFACE(3,2,((#252452,#252453,#252454),(#252455,#252456,#252457),
(#252458,#252459,#252460),(#252461,#252462,#252463)),.UNSPECIFIED.,.F.,
 .F.,.F.)
B_SPLINE_SURFACE_WITH_KNOTS((4,4),(3,3),(0.,0.000511815072430404),(0.,1.00105598365879),
 .UNSPECIFIED.)
GEOMETRIC_REPRESENTATION_ITEM()
RATIONAL_B_SPLINE_SURFACE(((1.,0.706797490733712,1.000619234117),(1.,0.706182062146633,
1.00062053388207),(1.,0.705584062768981,1.00062179683721),(1.,0.705266224770493,
1.00062246810067)))
REPRESENTATION_ITEM('')
SURFACE()
);
#3894=(
BOUNDED_SURFACE()
B_SPLINE_SURFACE(3,2,((#252469,#252470,#252471),(#252472,#252473,#252474),
(#252475,#252476,#252477),(#252478,#252479,#252480),(#252481,#252482,#252483),
(#252484,#252485,#252486)),.UNSPECIFIED.,.F.,.F.,.F.)
B_SPLINE_SURFACE_WITH_KNOTS((4,2,4),(3,3),(0.,0.000257652232350885,0.000515304464701769),
(0.,1.),.UNSPECIFIED.)
GEOMETRIC_REPRESENTATION_ITEM()
RATIONAL_B_SPLINE_SURFACE(((1.,0.87461970713938,1.),(1.,0.874861180430577,
1.),(1.,0.855455725921031,1.),(1.,0.794699358955064,1.),(1.,0.753768977788782,
1.),(1.,0.708712527163652,1.)))
REPRESENTATION_ITEM('')
SURFACE()
);
#3895=(
BOUNDED_SURFACE()
B_SPLINE_SURFACE(3,2,((#252492,#252493,#252494),(#252495,#252496,#252497),
(#252498,#252499,#252500),(#252501,#252502,#252503)),.UNSPECIFIED.,.F.,
 .F.,.F.)
B_SPLINE_SURFACE_WITH_KNOTS((4,4),(3,3),(0.,0.000397394373651918),(0.,1.),
 .UNSPECIFIED.)
GEOMETRIC_REPRESENTATION_ITEM()
RATIONAL_B_SPLINE_SURFACE(((1.,0.707106781186561,1.),(1.,0.707752587915879,
1.),(1.,0.708377654540666,1.),(1.,0.708689770883339,1.)))
REPRESENTATION_ITEM('')
SURFACE()
);
#3896=(
BOUNDED_SURFACE()
B_SPLINE_SURFACE(3,2,((#252505,#252506,#252507),(#252508,#252509,#252510),
(#252511,#252512,#252513),(#252514,#252515,#252516)),.UNSPECIFIED.,.F.,
 .F.,.F.)
B_SPLINE_SURFACE_WITH_KNOTS((4,4),(3,3),(0.,0.000511815456479793),(0.,1.00105873159869),
 .UNSPECIFIED.)
GEOMETRIC_REPRESENTATION_ITEM()
RATIONAL_B_SPLINE_SURFACE(((1.,0.708394529056689,1.00061746385288),(1.,
0.70805856416725,1.00061817524616),(1.,0.707430835372447,1.00061950443879),
(1.,0.706796685880741,1.000620847227)))
REPRESENTATION_ITEM('')
SURFACE()
);
#3897=(
BOUNDED_SURFACE()
B_SPLINE_SURFACE(3,2,((#252522,#252523,#252524),(#252525,#252526,#252527),
(#252528,#252529,#252530),(#252531,#252532,#252533)),.UNSPECIFIED.,.F.,
 .F.,.F.)
B_SPLINE_SURFACE_WITH_KNOTS((4,4),(3,3),(-5.96311194867027E-19,0.00039739446544832),
(0.,1.),.UNSPECIFIED.)
GEOMETRIC_REPRESENTATION_ITEM()
RATIONAL_B_SPLINE_SURFACE(((1.,0.705498956110792,1.),(1.,0.705821764811748,
1.),(1.,0.706461952521157,1.),(1.,0.70710678118655,1.)))
REPRESENTATION_ITEM('')
SURFACE()
);
#3898=(
BOUNDED_SURFACE()
B_SPLINE_SURFACE(3,2,((#252539,#252540,#252541),(#252542,#252543,#252544),
(#252545,#252546,#252547),(#252548,#252549,#252550)),.UNSPECIFIED.,.F.,
 .F.,.F.)
B_SPLINE_SURFACE_WITH_KNOTS((4,4),(3,3),(4.87890977618477E-19,0.000397394410828737),
(0.,1.),.UNSPECIFIED.)
GEOMETRIC_REPRESENTATION_ITEM()
RATIONAL_B_SPLINE_SURFACE(((1.,0.708689770883312,1.),(1.,0.708376440034555,
1.),(1.,0.707750498698384,1.),(1.,0.707106781186545,1.)))
REPRESENTATION_ITEM('')
SURFACE()
);
#3899=(
BOUNDED_SURFACE()
B_SPLINE_SURFACE(3,2,((#252556,#252557,#252558),(#252559,#252560,#252561),
(#252562,#252563,#252564),(#252565,#252566,#252567)),.UNSPECIFIED.,.F.,
 .F.,.F.)
B_SPLINE_SURFACE_WITH_KNOTS((4,4),(3,3),(0.,0.000511815090126186),(0.,1.00105592270295),
 .UNSPECIFIED.)
GEOMETRIC_REPRESENTATION_ITEM()
RATIONAL_B_SPLINE_SURFACE(((1.,0.705266242717264,1.00062243213128),(1.,
0.705584085908904,1.0006217608956),(1.,0.706182089450258,1.00062049800456),
(1.,0.706797508587261,1.00061919833449)))
REPRESENTATION_ITEM('')
SURFACE()
);
#3900=(
BOUNDED_SURFACE()
B_SPLINE_SURFACE(3,2,((#252569,#252570,#252571),(#252572,#252573,#252574),
(#252575,#252576,#252577),(#252578,#252579,#252580)),.UNSPECIFIED.,.F.,
 .F.,.F.)
B_SPLINE_SURFACE_WITH_KNOTS((4,4),(3,3),(-7.83336069620777E-18,0.000397394428086622),
(0.,1.),.UNSPECIFIED.)
GEOMETRIC_REPRESENTATION_ITEM()
RATIONAL_B_SPLINE_SURFACE(((1.,0.707106781186536,1.),(1.,0.70645984675912,
1.),(1.,0.705820510737251,1.),(1.,0.70549895611074,1.)))
REPRESENTATION_ITEM('')
SURFACE()
);
#3901=(
BOUNDED_SURFACE()
B_SPLINE_SURFACE(3,2,((#252586,#252587,#252588),(#252589,#252590,#252591),
(#252592,#252593,#252594),(#252595,#252596,#252597),(#252598,#252599,#252600),
(#252601,#252602,#252603)),.UNSPECIFIED.,.F.,.F.,.F.)
B_SPLINE_SURFACE_WITH_KNOTS((4,2,4),(3,3),(0.,0.000257953807872848,0.000515907615745697),
(0.,1.),.UNSPECIFIED.)
GEOMETRIC_REPRESENTATION_ITEM()
RATIONAL_B_SPLINE_SURFACE(((1.,0.874619707139394,1.),(1.,0.874834349679261,
1.),(1.,0.854686104157444,1.),(1.,0.792476597915463,1.),(1.,0.75088785459489,
1.),(1.,0.705585838031425,1.)))
REPRESENTATION_ITEM('')
SURFACE()
);
#3902=(
BOUNDED_SURFACE()
B_SPLINE_SURFACE(3,2,((#252609,#252610,#252611),(#252612,#252613,#252614),
(#252615,#252616,#252617),(#252618,#252619,#252620)),.UNSPECIFIED.,.F.,
 .F.,.F.)
B_SPLINE_SURFACE_WITH_KNOTS((4,4),(3,3),(0.,0.000511815437699154),(0.,1.00105881331701),
 .UNSPECIFIED.)
GEOMETRIC_REPRESENTATION_ITEM()
RATIONAL_B_SPLINE_SURFACE(((1.,0.706796661945988,1.00062089519784),(1.,
0.707430821224899,1.00061955228526),(1.,0.708058545830382,1.00061822299892),
(1.,0.708394505252395,1.0006175115623)))
REPRESENTATION_ITEM('')
SURFACE()
);
#3903=(
BOUNDED_SURFACE()
B_SPLINE_SURFACE(3,2,((#252622,#252623,#252624),(#252625,#252626,#252627),
(#252628,#252629,#252630),(#252631,#252632,#252633),(#252634,#252635,#252636),
(#252637,#252638,#252639)),.UNSPECIFIED.,.F.,.F.,.F.)
B_SPLINE_SURFACE_WITH_KNOTS((4,2,4),(3,3),(-1.35525271560688E-18,0.000256915317531253,
0.000513830635062508),(0.,1.),.UNSPECIFIED.)
GEOMETRIC_REPRESENTATION_ITEM()
RATIONAL_B_SPLINE_SURFACE(((1.,0.705585838031429,1.),(1.,0.750902433542525,
1.),(1.,0.792329530082822,1.),(1.,0.854288401593897,1.),(1.,0.874998031125356,
1.),(1.,0.87461970713939,1.)))
REPRESENTATION_ITEM('')
SURFACE()
);
#3904=(
BOUNDED_SURFACE()
B_SPLINE_SURFACE(3,2,((#252645,#252646,#252647),(#252648,#252649,#252650),
(#252651,#252652,#252653),(#252654,#252655,#252656),(#252657,#252658,#252659),
(#252660,#252661,#252662)),.UNSPECIFIED.,.F.,.F.,.F.)
B_SPLINE_SURFACE_WITH_KNOTS((4,2,4),(3,3),(-5.06864515636973E-18,0.000256592814262158,
0.00051318562852432),(0.,1.),.UNSPECIFIED.)
GEOMETRIC_REPRESENTATION_ITEM()
RATIONAL_B_SPLINE_SURFACE(((1.,0.708712527163671,1.),(1.,0.753780902613968,
1.),(1.,0.794538995768688,1.),(1.,0.855070770331595,1.),(1.,0.87501842744497,
1.),(1.,0.874619707139396,1.)))
REPRESENTATION_ITEM('')
SURFACE()
);
#3905=(
BOUNDED_SURFACE()
B_SPLINE_SURFACE(3,2,((#252664,#252665,#252666),(#252667,#252668,#252669),
(#252670,#252671,#252672),(#252673,#252674,#252675)),.UNSPECIFIED.,.F.,
 .F.,.F.)
B_SPLINE_SURFACE_WITH_KNOTS((4,4),(3,3),(0.,0.000511815072430407),(0.,1.0010559836599),
 .UNSPECIFIED.)
GEOMETRIC_REPRESENTATION_ITEM()
RATIONAL_B_SPLINE_SURFACE(((1.,0.706797490733387,1.00061923411766),(1.,
0.706182062146288,1.00062053388272),(1.,0.705584062768689,1.00062179683786),
(1.,0.705266224770146,1.00062246810133)))
REPRESENTATION_ITEM('')
SURFACE()
);
#3906=(
BOUNDED_SURFACE()
B_SPLINE_SURFACE(3,2,((#252681,#252682,#252683),(#252684,#252685,#252686),
(#252687,#252688,#252689),(#252690,#252691,#252692),(#252693,#252694,#252695),
(#252696,#252697,#252698)),.UNSPECIFIED.,.F.,.F.,.F.)
B_SPLINE_SURFACE_WITH_KNOTS((4,2,4),(3,3),(-3.06287113727155E-18,0.000257652232350878,
0.000515304464701758),(0.,1.),.UNSPECIFIED.)
GEOMETRIC_REPRESENTATION_ITEM()
RATIONAL_B_SPLINE_SURFACE(((1.,0.874619707139395,1.),(1.,0.874861180430859,
1.),(1.,0.85545572592067,1.),(1.,0.794699358955482,1.),(1.,0.753768977788507,
1.),(1.,0.708712527163654,1.)))
REPRESENTATION_ITEM('')
SURFACE()
);
#3907=(
BOUNDED_SURFACE()
B_SPLINE_SURFACE(3,2,((#252704,#252705,#252706),(#252707,#252708,#252709),
(#252710,#252711,#252712),(#252713,#252714,#252715)),.UNSPECIFIED.,.F.,
 .F.,.F.)
B_SPLINE_SURFACE_WITH_KNOTS((4,4),(3,3),(0.,0.000397394373651927),(0.,1.),
 .UNSPECIFIED.)
GEOMETRIC_REPRESENTATION_ITEM()
RATIONAL_B_SPLINE_SURFACE(((1.,0.707106781186541,1.),(1.,0.707752587915892,
1.),(1.,0.708377654540697,1.),(1.,0.708689770883313,1.)))
REPRESENTATION_ITEM('')
SURFACE()
);
#3908=(
BOUNDED_SURFACE()
B_SPLINE_SURFACE(3,2,((#252717,#252718,#252719),(#252720,#252721,#252722),
(#252723,#252724,#252725),(#252726,#252727,#252728)),.UNSPECIFIED.,.F.,
 .F.,.F.)
B_SPLINE_SURFACE_WITH_KNOTS((4,4),(3,3),(0.,0.000511815456479792),(0.,1.0010587316),
 .UNSPECIFIED.)
GEOMETRIC_REPRESENTATION_ITEM()
RATIONAL_B_SPLINE_SURFACE(((1.,0.708394529056316,1.00061746385364),(1.,
0.708058564166859,1.00061817524693),(1.,0.707430835372039,1.00061950443955),
(1.,0.706796685880368,1.00062084722776)))
REPRESENTATION_ITEM('')
SURFACE()
);
#3909=(
BOUNDED_SURFACE()
B_SPLINE_SURFACE(3,2,((#252734,#252735,#252736),(#252737,#252738,#252739),
(#252740,#252741,#252742),(#252743,#252744,#252745)),.UNSPECIFIED.,.F.,
 .F.,.F.)
B_SPLINE_SURFACE_WITH_KNOTS((4,4),(3,3),(-6.20705743747951E-18,0.000397394465448313),
(0.,1.),.UNSPECIFIED.)
GEOMETRIC_REPRESENTATION_ITEM()
RATIONAL_B_SPLINE_SURFACE(((1.,0.705498956110768,1.),(1.,0.705821764811784,
1.),(1.,0.706461952521158,1.),(1.,0.707106781186533,1.)))
REPRESENTATION_ITEM('')
SURFACE()
);
#3910=(
BOUNDED_SURFACE()
B_SPLINE_SURFACE(3,2,((#252751,#252752,#252753),(#252754,#252755,#252756),
(#252757,#252758,#252759),(#252760,#252761,#252762)),.UNSPECIFIED.,.F.,
 .F.,.F.)
B_SPLINE_SURFACE_WITH_KNOTS((4,4),(3,3),(3.52365706057789E-19,0.000397394410828728),
(0.,1.),.UNSPECIFIED.)
GEOMETRIC_REPRESENTATION_ITEM()
RATIONAL_B_SPLINE_SURFACE(((1.,0.708689770883317,1.),(1.,0.708376440034512,
1.),(1.,0.707750498698386,1.),(1.,0.707106781186551,1.)))
REPRESENTATION_ITEM('')
SURFACE()
);
#3911=(
BOUNDED_SURFACE()
B_SPLINE_SURFACE(3,2,((#252768,#252769,#252770),(#252771,#252772,#252773),
(#252774,#252775,#252776),(#252777,#252778,#252779)),.UNSPECIFIED.,.F.,
 .F.,.F.)
B_SPLINE_SURFACE_WITH_KNOTS((4,4),(3,3),(0.,0.000511815090126187),(0.,1.00105592270218),
 .UNSPECIFIED.)
GEOMETRIC_REPRESENTATION_ITEM()
RATIONAL_B_SPLINE_SURFACE(((1.,0.705266242717496,1.00062243213083),(1.,
0.705584085909148,1.00062176089515),(1.,0.706182089450495,1.00062049800412),
(1.,0.70679750858749,1.00061919833404)))
REPRESENTATION_ITEM('')
SURFACE()
);
#3912=(
BOUNDED_SURFACE()
B_SPLINE_SURFACE(3,2,((#252781,#252782,#252783),(#252784,#252785,#252786),
(#252787,#252788,#252789),(#252790,#252791,#252792)),.UNSPECIFIED.,.F.,
 .F.,.F.)
B_SPLINE_SURFACE_WITH_KNOTS((4,4),(3,3),(0.,0.00039739442808662),(0.,1.),
 .UNSPECIFIED.)
GEOMETRIC_REPRESENTATION_ITEM()
RATIONAL_B_SPLINE_SURFACE(((1.,0.707106781186551,1.),(1.,0.706459846759092,
1.),(1.,0.705820510737283,1.),(1.,0.705498956110754,1.)))
REPRESENTATION_ITEM('')
SURFACE()
);
#3913=(
BOUNDED_SURFACE()
B_SPLINE_SURFACE(3,2,((#252798,#252799,#252800),(#252801,#252802,#252803),
(#252804,#252805,#252806),(#252807,#252808,#252809),(#252810,#252811,#252812),
(#252813,#252814,#252815)),.UNSPECIFIED.,.F.,.F.,.F.)
B_SPLINE_SURFACE_WITH_KNOTS((4,2,4),(3,3),(-3.27971157176865E-18,0.00025795380787285,
0.000515907615745704),(0.,1.),.UNSPECIFIED.)
GEOMETRIC_REPRESENTATION_ITEM()
RATIONAL_B_SPLINE_SURFACE(((1.,0.874619707139389,1.),(1.,0.874834349679203,
1.),(1.,0.854686104157534,1.),(1.,0.792476597915407,1.),(1.,0.750887854594928,
1.),(1.,0.705585838031446,1.)))
REPRESENTATION_ITEM('')
SURFACE()
);
#3914=(
BOUNDED_SURFACE()
B_SPLINE_SURFACE(3,2,((#252821,#252822,#252823),(#252824,#252825,#252826),
(#252827,#252828,#252829),(#252830,#252831,#252832)),.UNSPECIFIED.,.F.,
 .F.,.F.)
B_SPLINE_SURFACE_WITH_KNOTS((4,4),(3,3),(0.,0.000511815437699159),(0.,1.00105881331807),
 .UNSPECIFIED.)
GEOMETRIC_REPRESENTATION_ITEM()
RATIONAL_B_SPLINE_SURFACE(((1.,0.706796661945702,1.00062089519847),(1.,
0.707430821224571,1.00061955228589),(1.,0.70805854583007,1.00061822299954),
(1.,0.708394505252093,1.00061751156292)))
REPRESENTATION_ITEM('')
SURFACE()
);
#3915=(
BOUNDED_SURFACE()
B_SPLINE_SURFACE(3,2,((#252834,#252835,#252836),(#252837,#252838,#252839),
(#252840,#252841,#252842),(#252843,#252844,#252845),(#252846,#252847,#252848),
(#252849,#252850,#252851)),.UNSPECIFIED.,.F.,.F.,.F.)
B_SPLINE_SURFACE_WITH_KNOTS((4,2,4),(3,3),(-1.13841228110978E-18,0.00025691531753126,
0.000513830635062521),(0.,1.),.UNSPECIFIED.)
GEOMETRIC_REPRESENTATION_ITEM()
RATIONAL_B_SPLINE_SURFACE(((1.,0.705585838031441,1.),(1.,0.750902433542694,
1.),(1.,0.792329530082573,1.),(1.,0.854288401594117,1.),(1.,0.87499803112519,
1.),(1.,0.874619707139408,1.)))
REPRESENTATION_ITEM('')
SURFACE()
);
#3916=(
BOUNDED_SURFACE()
B_SPLINE_SURFACE(3,2,((#252857,#252858,#252859),(#252860,#252861,#252862),
(#252863,#252864,#252865),(#252866,#252867,#252868),(#252869,#252870,#252871),
(#252872,#252873,#252874)),.UNSPECIFIED.,.F.,.F.,.F.)
B_SPLINE_SURFACE_WITH_KNOTS((4,2,4),(3,3),(-2.0870891820346E-18,0.000256592814262156,
0.000513185628524313),(0.,1.),.UNSPECIFIED.)
GEOMETRIC_REPRESENTATION_ITEM()
RATIONAL_B_SPLINE_SURFACE(((1.,0.708712527163635,1.),(1.,0.753780902613681,
1.),(1.,0.794538995769107,1.),(1.,0.855070770331192,1.),(1.,0.875018427445252,
1.),(1.,0.874619707139401,1.)))
REPRESENTATION_ITEM('')
SURFACE()
);
#3917=(
BOUNDED_SURFACE()
B_SPLINE_SURFACE(3,2,((#252876,#252877,#252878),(#252879,#252880,#252881),
(#252882,#252883,#252884),(#252885,#252886,#252887)),.UNSPECIFIED.,.F.,
 .F.,.F.)
B_SPLINE_SURFACE_WITH_KNOTS((4,4),(3,3),(-7.77915058758349E-18,0.0005118150724304),
(0.,1.00105598365789),.UNSPECIFIED.)
GEOMETRIC_REPRESENTATION_ITEM()
RATIONAL_B_SPLINE_SURFACE(((1.,0.706797490733977,1.00061923411647),(1.,
0.706182062146854,1.00062053388153),(1.,0.705584062769277,1.00062179683667),
(1.,0.705266224770748,1.00062246810014)))
REPRESENTATION_ITEM('')
SURFACE()
);
#3918=(
BOUNDED_SURFACE()
B_SPLINE_SURFACE(3,2,((#252893,#252894,#252895),(#252896,#252897,#252898),
(#252899,#252900,#252901),(#252902,#252903,#252904),(#252905,#252906,#252907),
(#252908,#252909,#252910)),.UNSPECIFIED.,.F.,.F.,.F.)
B_SPLINE_SURFACE_WITH_KNOTS((4,2,4),(3,3),(-3.21194893598831E-18,0.000257652232350879,
0.000515304464701761),(0.,1.),.UNSPECIFIED.)
GEOMETRIC_REPRESENTATION_ITEM()
RATIONAL_B_SPLINE_SURFACE(((1.,0.874619707139399,1.),(1.,0.874861180430952,
1.),(1.,0.855455725920543,1.),(1.,0.794699358955585,1.),(1.,0.753768977788435,
1.),(1.,0.708712527163638,1.)))
REPRESENTATION_ITEM('')
SURFACE()
);
#3919=(
BOUNDED_SURFACE()
B_SPLINE_SURFACE(3,2,((#252916,#252917,#252918),(#252919,#252920,#252921),
(#252922,#252923,#252924),(#252925,#252926,#252927)),.UNSPECIFIED.,.F.,
 .F.,.F.)
B_SPLINE_SURFACE_WITH_KNOTS((4,4),(3,3),(-1.44740990026815E-17,0.000397394373651909),
(0.,1.),.UNSPECIFIED.)
GEOMETRIC_REPRESENTATION_ITEM()
RATIONAL_B_SPLINE_SURFACE(((1.,0.707106781186544,1.),(1.,0.70775258791589,
1.),(1.,0.708377654540694,1.),(1.,0.708689770883335,1.)))
REPRESENTATION_ITEM('')
SURFACE()
);
#3920=(
BOUNDED_SURFACE()
B_SPLINE_SURFACE(3,2,((#252929,#252930,#252931),(#252932,#252933,#252934),
(#252935,#252936,#252937),(#252938,#252939,#252940)),.UNSPECIFIED.,.F.,
 .F.,.F.)
B_SPLINE_SURFACE_WITH_KNOTS((4,4),(3,3),(-6.42389787197661E-18,0.000511815456479789),
(0.,1.00105873159907),.UNSPECIFIED.)
GEOMETRIC_REPRESENTATION_ITEM()
RATIONAL_B_SPLINE_SURFACE(((1.,0.708394529056584,1.0006174638531),(1.,0.708058564167148,
1.00061817524639),(1.,0.707430835372308,1.00061950443901),(1.,0.706796685880638,
1.00062084722722)))
REPRESENTATION_ITEM('')
SURFACE()
);
#3921=(
BOUNDED_SURFACE()
B_SPLINE_SURFACE(3,2,((#252946,#252947,#252948),(#252949,#252950,#252951),
(#252952,#252953,#252954),(#252955,#252956,#252957)),.UNSPECIFIED.,.F.,
 .F.,.F.)
B_SPLINE_SURFACE_WITH_KNOTS((4,4),(3,3),(-3.79470760369927E-19,0.000397394465448309),
(0.,1.),.UNSPECIFIED.)
GEOMETRIC_REPRESENTATION_ITEM()
RATIONAL_B_SPLINE_SURFACE(((1.,0.705498956110748,1.),(1.,0.705821764811732,
1.),(1.,0.706461952521157,1.),(1.,0.707106781186544,1.)))
REPRESENTATION_ITEM('')
SURFACE()
);
#3922=(
BOUNDED_SURFACE()
B_SPLINE_SURFACE(3,2,((#252963,#252964,#252965),(#252966,#252967,#252968),
(#252969,#252970,#252971),(#252972,#252973,#252974)),.UNSPECIFIED.,.F.,
 .F.,.F.)
B_SPLINE_SURFACE_WITH_KNOTS((4,4),(3,3),(0.,0.000397394410828749),(0.,1.),
 .UNSPECIFIED.)
GEOMETRIC_REPRESENTATION_ITEM()
RATIONAL_B_SPLINE_SURFACE(((1.,0.70868977088334,1.),(1.,0.708376440034472,
1.),(1.,0.707750498698436,1.),(1.,0.707106781186546,1.)))
REPRESENTATION_ITEM('')
SURFACE()
);
#3923=(
BOUNDED_SURFACE()
B_SPLINE_SURFACE(3,2,((#252980,#252981,#252982),(#252983,#252984,#252985),
(#252986,#252987,#252988),(#252989,#252990,#252991)),.UNSPECIFIED.,.F.,
 .F.,.F.)
B_SPLINE_SURFACE_WITH_KNOTS((4,4),(3,3),(-1.35525271560688E-19,0.000511815090126169),
(0.,1.00105592270159),.UNSPECIFIED.)
GEOMETRIC_REPRESENTATION_ITEM()
RATIONAL_B_SPLINE_SURFACE(((1.,0.705266242717656,1.00062243213048),(1.,
0.705584085909313,1.0006217608948),(1.,0.706182089450677,1.00062049800377),
(1.,0.706797508587662,1.00061919833369)))
REPRESENTATION_ITEM('')
SURFACE()
);
#3924=(
BOUNDED_SURFACE()
B_SPLINE_SURFACE(3,2,((#252993,#252994,#252995),(#252996,#252997,#252998),
(#252999,#253000,#253001),(#253002,#253003,#253004)),.UNSPECIFIED.,.F.,
 .F.,.F.)
B_SPLINE_SURFACE_WITH_KNOTS((4,4),(3,3),(0.,0.000397394428086617),(0.,1.),
 .UNSPECIFIED.)
GEOMETRIC_REPRESENTATION_ITEM()
RATIONAL_B_SPLINE_SURFACE(((1.,0.707106781186545,1.),(1.,0.706459846759076,
1.),(1.,0.705820510737292,1.),(1.,0.705498956110732,1.)))
REPRESENTATION_ITEM('')
SURFACE()
);
#3925=(
BOUNDED_SURFACE()
B_SPLINE_SURFACE(3,2,((#253010,#253011,#253012),(#253013,#253014,#253015),
(#253016,#253017,#253018),(#253019,#253020,#253021),(#253022,#253023,#253024),
(#253025,#253026,#253027)),.UNSPECIFIED.,.F.,.F.,.F.)
B_SPLINE_SURFACE_WITH_KNOTS((4,2,4),(3,3),(-5.14996031930615E-19,0.000257953807872849,
0.000515907615745698),(0.,1.),.UNSPECIFIED.)
GEOMETRIC_REPRESENTATION_ITEM()
RATIONAL_B_SPLINE_SURFACE(((1.,0.874619707139401,1.),(1.,0.874834349678968,
1.),(1.,0.85468610415782,1.),(1.,0.792476597915128,1.),(1.,0.750887854595128,
1.),(1.,0.70558583803143,1.)))
REPRESENTATION_ITEM('')
SURFACE()
);
#3926=(
BOUNDED_SURFACE()
B_SPLINE_SURFACE(3,2,((#253033,#253034,#253035),(#253036,#253037,#253038),
(#253039,#253040,#253041),(#253042,#253043,#253044)),.UNSPECIFIED.,.F.,
 .F.,.F.)
B_SPLINE_SURFACE_WITH_KNOTS((4,4),(3,3),(-8.13151629364128E-20,0.000511815437699142),
(0.,1.00105881331387),.UNSPECIFIED.)
GEOMETRIC_REPRESENTATION_ITEM()
RATIONAL_B_SPLINE_SURFACE(((1.,0.706796661946928,1.000620895196),(1.,0.707430821225802,
1.00061955228343),(1.,0.708058545831284,1.00061822299709),(1.,0.708394505253304,
1.00061751156047)))
REPRESENTATION_ITEM('')
SURFACE()
);
#3927=(
BOUNDED_SURFACE()
B_SPLINE_SURFACE(3,2,((#253046,#253047,#253048),(#253049,#253050,#253051),
(#253052,#253053,#253054),(#253055,#253056,#253057),(#253058,#253059,#253060),
(#253061,#253062,#253063)),.UNSPECIFIED.,.F.,.F.,.F.)
B_SPLINE_SURFACE_WITH_KNOTS((4,2,4),(3,3),(-4.49943901581484E-18,0.000256915317531251,
0.000513830635062507),(0.,1.),.UNSPECIFIED.)
GEOMETRIC_REPRESENTATION_ITEM()
RATIONAL_B_SPLINE_SURFACE(((1.,0.705585838031437,1.),(1.,0.750902433542874,
1.),(1.,0.79232953008234,1.),(1.,0.854288401594352,1.),(1.,0.874998031125028,
1.),(1.,0.874619707139391,1.)))
REPRESENTATION_ITEM('')
SURFACE()
);
#3928=(
BOUNDED_SURFACE()
B_SPLINE_SURFACE(3,2,((#253069,#253070,#253071),(#253072,#253073,#253074),
(#253075,#253076,#253077),(#253078,#253079,#253080),(#253081,#253082,#253083),
(#253084,#253085,#253086)),.UNSPECIFIED.,.F.,.F.,.F.)
B_SPLINE_SURFACE_WITH_KNOTS((4,2,4),(3,3),(-3.25260651745651E-19,0.000256592814262156,
0.000513185628524313),(0.,1.),.UNSPECIFIED.)
GEOMETRIC_REPRESENTATION_ITEM()
RATIONAL_B_SPLINE_SURFACE(((1.,0.708712527163664,1.),(1.,0.753780902612852,
1.),(1.,0.794538995770168,1.),(1.,0.855070770330182,1.),(1.,0.875018427446005,
1.),(1.,0.874619707139394,1.)))
REPRESENTATION_ITEM('')
SURFACE()
);
#3929=(
BOUNDED_SURFACE()
B_SPLINE_SURFACE(3,2,((#253088,#253089,#253090),(#253091,#253092,#253093),
(#253094,#253095,#253096),(#253097,#253098,#253099)),.UNSPECIFIED.,.F.,
 .F.,.F.)
B_SPLINE_SURFACE_WITH_KNOTS((4,4),(3,3),(2.71050543121376E-20,0.000511815072430397),
(0.,1.00105598365838),.UNSPECIFIED.)
GEOMETRIC_REPRESENTATION_ITEM()
RATIONAL_B_SPLINE_SURFACE(((1.,0.706797490733823,1.00061923411676),(1.,
0.706182062146751,1.00062053388183),(1.,0.705584062769127,1.00062179683697),
(1.,0.70526622477057,1.00062246810043)))
REPRESENTATION_ITEM('')
SURFACE()
);
#3930=(
BOUNDED_SURFACE()
B_SPLINE_SURFACE(3,2,((#253105,#253106,#253107),(#253108,#253109,#253110),
(#253111,#253112,#253113),(#253114,#253115,#253116),(#253117,#253118,#253119),
(#253120,#253121,#253122)),.UNSPECIFIED.,.F.,.F.,.F.)
B_SPLINE_SURFACE_WITH_KNOTS((4,2,4),(3,3),(0.,0.000257652232350884,0.000515304464701769),
(0.,1.),.UNSPECIFIED.)
GEOMETRIC_REPRESENTATION_ITEM()
RATIONAL_B_SPLINE_SURFACE(((1.,0.874619707139393,1.),(1.,0.874861180430782,
1.),(1.,0.85545572592081,1.),(1.,0.794699358955333,1.),(1.,0.753768977788603,
1.),(1.,0.708712527163673,1.)))
REPRESENTATION_ITEM('')
SURFACE()
);
#3931=(
BOUNDED_SURFACE()
B_SPLINE_SURFACE(3,2,((#253128,#253129,#253130),(#253131,#253132,#253133),
(#253134,#253135,#253136),(#253137,#253138,#253139)),.UNSPECIFIED.,.F.,
 .F.,.F.)
B_SPLINE_SURFACE_WITH_KNOTS((4,4),(3,3),(0.,0.000397394373651932),(0.,1.),
 .UNSPECIFIED.)
GEOMETRIC_REPRESENTATION_ITEM()
RATIONAL_B_SPLINE_SURFACE(((1.,0.707106781186545,1.),(1.,0.707752587915885,
1.),(1.,0.708377654540695,1.),(1.,0.70868977088333,1.)))
REPRESENTATION_ITEM('')
SURFACE()
);
#3932=(
BOUNDED_SURFACE()
B_SPLINE_SURFACE(3,2,((#253141,#253142,#253143),(#253144,#253145,#253146),
(#253147,#253148,#253149),(#253150,#253151,#253152)),.UNSPECIFIED.,.F.,
 .F.,.F.)
B_SPLINE_SURFACE_WITH_KNOTS((4,4),(3,3),(1.35525271560688E-19,0.000511815456479789),
(0.,1.00105873159949),.UNSPECIFIED.)
GEOMETRIC_REPRESENTATION_ITEM()
RATIONAL_B_SPLINE_SURFACE(((1.,0.708394529056461,1.00061746385335),(1.,
0.708058564166996,1.00061817524664),(1.,0.707430835372202,1.00061950443926),
(1.,0.70679668588051,1.00062084722747)))
REPRESENTATION_ITEM('')
SURFACE()
);
#3933=(
BOUNDED_SURFACE()
B_SPLINE_SURFACE(3,2,((#253158,#253159,#253160),(#253161,#253162,#253163),
(#253164,#253165,#253166),(#253167,#253168,#253169)),.UNSPECIFIED.,.F.,
 .F.,.F.)
B_SPLINE_SURFACE_WITH_KNOTS((4,4),(3,3),(0.,0.000397394465448298),(0.,1.),
 .UNSPECIFIED.)
GEOMETRIC_REPRESENTATION_ITEM()
RATIONAL_B_SPLINE_SURFACE(((1.,0.705498956110754,1.),(1.,0.705821764811776,
1.),(1.,0.706461952521147,1.),(1.,0.707106781186545,1.)))
REPRESENTATION_ITEM('')
SURFACE()
);
#3934=(
BOUNDED_SURFACE()
B_SPLINE_SURFACE(3,2,((#253175,#253176,#253177),(#253178,#253179,#253180),
(#253181,#253182,#253183),(#253184,#253185,#253186)),.UNSPECIFIED.,.F.,
 .F.,.F.)
B_SPLINE_SURFACE_WITH_KNOTS((4,4),(3,3),(2.71050543121376E-20,0.000397394410828729),
(0.,1.),.UNSPECIFIED.)
GEOMETRIC_REPRESENTATION_ITEM()
RATIONAL_B_SPLINE_SURFACE(((1.,0.70868977088331,1.),(1.,0.708376440034508,
1.),(1.,0.707750498698394,1.),(1.,0.707106781186548,1.)))
REPRESENTATION_ITEM('')
SURFACE()
);
#3935=(
BOUNDED_SURFACE()
B_SPLINE_SURFACE(3,2,((#253192,#253193,#253194),(#253195,#253196,#253197),
(#253198,#253199,#253200),(#253201,#253202,#253203)),.UNSPECIFIED.,.F.,
 .F.,.F.)
B_SPLINE_SURFACE_WITH_KNOTS((4,4),(3,3),(-2.71050543121376E-20,0.000511815090126182),
(0.,1.00105592270603),.UNSPECIFIED.)
GEOMETRIC_REPRESENTATION_ITEM()
RATIONAL_B_SPLINE_SURFACE(((1.,0.705266242716357,1.0006224321331),(1.,0.705584085908022,
1.00062176089741),(1.,0.706182089449371,1.00062049800638),(1.,0.706797508586361,
1.0006191983363)))
REPRESENTATION_ITEM('')
SURFACE()
);
#3936=(
BOUNDED_SURFACE()
B_SPLINE_SURFACE(3,2,((#253205,#253206,#253207),(#253208,#253209,#253210),
(#253211,#253212,#253213),(#253214,#253215,#253216)),.UNSPECIFIED.,.F.,
 .F.,.F.)
B_SPLINE_SURFACE_WITH_KNOTS((4,4),(3,3),(1.0842021724855E-19,0.00039739442808663),
(0.,1.),.UNSPECIFIED.)
GEOMETRIC_REPRESENTATION_ITEM()
RATIONAL_B_SPLINE_SURFACE(((1.,0.70710678118655,1.),(1.,0.706459846759098,
1.),(1.,0.705820510737275,1.),(1.,0.705498956110757,1.)))
REPRESENTATION_ITEM('')
SURFACE()
);
#3937=(
BOUNDED_SURFACE()
B_SPLINE_SURFACE(3,2,((#253222,#253223,#253224),(#253225,#253226,#253227),
(#253228,#253229,#253230),(#253231,#253232,#253233),(#253234,#253235,#253236),
(#253237,#253238,#253239)),.UNSPECIFIED.,.F.,.F.,.F.)
B_SPLINE_SURFACE_WITH_KNOTS((4,2,4),(3,3),(0.,0.00025795380787284,0.00051590761574568),
(0.,1.),.UNSPECIFIED.)
GEOMETRIC_REPRESENTATION_ITEM()
RATIONAL_B_SPLINE_SURFACE(((1.,0.87461970713939,1.),(1.,0.874834349678797,
1.),(1.,0.854686104158041,1.),(1.,0.792476597914909,1.),(1.,0.750887854595297,
1.),(1.,0.705585838031443,1.)))
REPRESENTATION_ITEM('')
SURFACE()
);
#3938=(
BOUNDED_SURFACE()
B_SPLINE_SURFACE(3,2,((#253245,#253246,#253247),(#253248,#253249,#253250),
(#253251,#253252,#253253),(#253254,#253255,#253256)),.UNSPECIFIED.,.F.,
 .F.,.F.)
B_SPLINE_SURFACE_WITH_KNOTS((4,4),(3,3),(-7.23704950134074E-18,0.000511815437699144),
(0.,1.00105881331707),.UNSPECIFIED.)
GEOMETRIC_REPRESENTATION_ITEM()
RATIONAL_B_SPLINE_SURFACE(((1.,0.706796661945989,1.00062089519788),(1.,
0.70743082122485,1.0006195522853),(1.,0.708058545830382,1.00061822299896),
(1.,0.708394505252367,1.00061751156234)))
REPRESENTATION_ITEM('')
SURFACE()
);
#3939=(
BOUNDED_SURFACE()
B_SPLINE_SURFACE(3,2,((#253258,#253259,#253260),(#253261,#253262,#253263),
(#253264,#253265,#253266),(#253267,#253268,#253269),(#253270,#253271,#253272),
(#253273,#253274,#253275)),.UNSPECIFIED.,.F.,.F.,.F.)
B_SPLINE_SURFACE_WITH_KNOTS((4,2,4),(3,3),(-2.43945488809238E-19,0.00025691531753126,
0.00051383063506252),(0.,1.),.UNSPECIFIED.)
GEOMETRIC_REPRESENTATION_ITEM()
RATIONAL_B_SPLINE_SURFACE(((1.,0.705585838031451,1.),(1.,0.750902433542877,
1.),(1.,0.792329530082299,1.),(1.,0.854288401594406,1.),(1.,0.874998031124972,
1.),(1.,0.874619707139391,1.)))
REPRESENTATION_ITEM('')
SURFACE()
);
#3940=(
BOUNDED_SURFACE()
B_SPLINE_SURFACE(3,2,((#253281,#253282,#253283),(#253284,#253285,#253286),
(#253287,#253288,#253289),(#253290,#253291,#253292),(#253293,#253294,#253295),
(#253296,#253297,#253298)),.UNSPECIFIED.,.F.,.F.,.F.)
B_SPLINE_SURFACE_WITH_KNOTS((4,2,4),(3,3),(1.89735380184963E-19,0.000256592814262156,
0.000513185628524311),(0.,1.),.UNSPECIFIED.)
GEOMETRIC_REPRESENTATION_ITEM()
RATIONAL_B_SPLINE_SURFACE(((1.,0.708712527163678,1.),(1.,0.753780902613698,
1.),(1.,0.794538995769049,1.),(1.,0.855070770331267,1.),(1.,0.875018427445209,
1.),(1.,0.874619707139396,1.)))
REPRESENTATION_ITEM('')
SURFACE()
);
#3941=(
BOUNDED_SURFACE()
B_SPLINE_SURFACE(3,2,((#253300,#253301,#253302),(#253303,#253304,#253305),
(#253306,#253307,#253308),(#253309,#253310,#253311)),.UNSPECIFIED.,.F.,
 .F.,.F.)
B_SPLINE_SURFACE_WITH_KNOTS((4,4),(3,3),(-4.87890977618477E-19,0.000511815072430402),
(0.,1.001055983659),.UNSPECIFIED.)
GEOMETRIC_REPRESENTATION_ITEM()
RATIONAL_B_SPLINE_SURFACE(((1.,0.706797490733651,1.00061923411713),(1.,
0.706182062146538,1.00062053388219),(1.,0.705584062768948,1.00062179683733),
(1.,0.705266224770404,1.0006224681008)))
REPRESENTATION_ITEM('')
SURFACE()
);
#3942=(
BOUNDED_SURFACE()
B_SPLINE_SURFACE(3,2,((#253317,#253318,#253319),(#253320,#253321,#253322),
(#253323,#253324,#253325),(#253326,#253327,#253328),(#253329,#253330,#253331),
(#253332,#253333,#253334)),.UNSPECIFIED.,.F.,.F.,.F.)
B_SPLINE_SURFACE_WITH_KNOTS((4,2,4),(3,3),(-3.11708124589583E-19,0.00025765223235088,
0.00051530446470176),(0.,1.),.UNSPECIFIED.)
GEOMETRIC_REPRESENTATION_ITEM()
RATIONAL_B_SPLINE_SURFACE(((1.,0.874619707139394,1.),(1.,0.874861180430961,
1.),(1.,0.855455725920548,1.),(1.,0.794699358955591,1.),(1.,0.75376897778842,
1.),(1.,0.70871252716367,1.)))
REPRESENTATION_ITEM('')
SURFACE()
);
#3943=(
BOUNDED_SURFACE()
B_SPLINE_SURFACE(3,2,((#253340,#253341,#253342),(#253343,#253344,#253345),
(#253346,#253347,#253348),(#253349,#253350,#253351)),.UNSPECIFIED.,.F.,
 .F.,.F.)
B_SPLINE_SURFACE_WITH_KNOTS((4,4),(3,3),(-8.13151629364128E-20,0.000397394373651932),
(0.,1.),.UNSPECIFIED.)
GEOMETRIC_REPRESENTATION_ITEM()
RATIONAL_B_SPLINE_SURFACE(((1.,0.707106781186547,1.),(1.,0.707752587915892,
1.),(1.,0.708377654540687,1.),(1.,0.708689770883334,1.)))
REPRESENTATION_ITEM('')
SURFACE()
);
#3944=(
BOUNDED_SURFACE()
B_SPLINE_SURFACE(3,2,((#253353,#253354,#253355),(#253356,#253357,#253358),
(#253359,#253360,#253361),(#253362,#253363,#253364)),.UNSPECIFIED.,.F.,
 .F.,.F.)
B_SPLINE_SURFACE_WITH_KNOTS((4,4),(3,3),(2.71050543121376E-20,0.000511815456479785),
(0.,1.00105873159858),.UNSPECIFIED.)
GEOMETRIC_REPRESENTATION_ITEM()
RATIONAL_B_SPLINE_SURFACE(((1.,0.708394529056732,1.00061746385281),(1.,
0.708058564167282,1.0006181752461),(1.,0.707430835372459,1.00061950443872),
(1.,0.706796685880782,1.00062084722693)))
REPRESENTATION_ITEM('')
SURFACE()
);
#3945=(
BOUNDED_SURFACE()
B_SPLINE_SURFACE(3,2,((#253370,#253371,#253372),(#253373,#253374,#253375),
(#253376,#253377,#253378),(#253379,#253380,#253381)),.UNSPECIFIED.,.F.,
 .F.,.F.)
B_SPLINE_SURFACE_WITH_KNOTS((4,4),(3,3),(-2.71050543121376E-20,0.000397394465448309),
(0.,1.),.UNSPECIFIED.)
GEOMETRIC_REPRESENTATION_ITEM()
RATIONAL_B_SPLINE_SURFACE(((1.,0.705498956110728,1.),(1.,0.705821764811776,
1.),(1.,0.706461952521145,1.),(1.,0.707106781186548,1.)))
REPRESENTATION_ITEM('')
SURFACE()
);
#3946=(
BOUNDED_SURFACE()
B_SPLINE_SURFACE(2,2,((#253474,#253475,#253476),(#253477,#253478,#253479),
(#253480,#253481,#253482)),.UNSPECIFIED.,.F.,.F.,.F.)
B_SPLINE_SURFACE_WITH_KNOTS((3,3),(3,3),(-1.5707963267949,0.),(-0.314644728766082,
0.610865238198018),.UNSPECIFIED.)
GEOMETRIC_REPRESENTATION_ITEM()
RATIONAL_B_SPLINE_SURFACE(((1.,0.894826028883616,1.),(0.707106781186549,
0.632737553005835,0.707106781186549),(1.,0.894826028883616,1.)))
REPRESENTATION_ITEM('')
SURFACE()
);
#3947=(
BOUNDED_SURFACE()
B_SPLINE_SURFACE(2,2,((#253491,#253492,#253493),(#253494,#253495,#253496),
(#253497,#253498,#253499)),.UNSPECIFIED.,.F.,.F.,.F.)
B_SPLINE_SURFACE_WITH_KNOTS((3,3),(3,3),(-1.5707963267949,0.),(-0.610865238198018,
0.314644728766082),.UNSPECIFIED.)
GEOMETRIC_REPRESENTATION_ITEM()
RATIONAL_B_SPLINE_SURFACE(((1.,0.894826028883616,1.),(0.707106781186549,
0.632737553005836,0.707106781186549),(1.,0.894826028883616,1.)))
REPRESENTATION_ITEM('')
SURFACE()
);
#3948=(
BOUNDED_SURFACE()
B_SPLINE_SURFACE(2,2,((#253508,#253509,#253510),(#253511,#253512,#253513),
(#253514,#253515,#253516)),.UNSPECIFIED.,.F.,.F.,.F.)
B_SPLINE_SURFACE_WITH_KNOTS((3,3),(3,3),(-1.5707963267949,0.),(-0.462754983482051,
0.462754983482052),.UNSPECIFIED.)
GEOMETRIC_REPRESENTATION_ITEM()
RATIONAL_B_SPLINE_SURFACE(((1.,0.894826028883615,1.),(0.707106781186545,
0.632737553005831,0.707106781186545),(1.,0.894826028883615,1.)))
REPRESENTATION_ITEM('')
SURFACE()
);
#3949=(
BOUNDED_SURFACE()
B_SPLINE_SURFACE(2,2,((#253531,#253532,#253533),(#253534,#253535,#253536),
(#253537,#253538,#253539)),.UNSPECIFIED.,.F.,.F.,.F.)
B_SPLINE_SURFACE_WITH_KNOTS((3,3),(3,3),(-1.5707963267949,0.),(-0.462754983482049,
0.46275498348205),.UNSPECIFIED.)
GEOMETRIC_REPRESENTATION_ITEM()
RATIONAL_B_SPLINE_SURFACE(((1.,0.894826028883616,1.),(0.707106781186543,
0.63273755300583,0.707106781186543),(1.,0.894826028883616,1.)))
REPRESENTATION_ITEM('')
SURFACE()
);
#3950=(
BOUNDED_SURFACE()
B_SPLINE_SURFACE(3,1,((#254918,#254919),(#254920,#254921),(#254922,#254923),
(#254924,#254925)),.UNSPECIFIED.,.F.,.F.,.F.)
B_SPLINE_SURFACE_WITH_KNOTS((4,4),(2,2),(0.,1.),(0.,1.),.UNSPECIFIED.)
GEOMETRIC_REPRESENTATION_ITEM()
RATIONAL_B_SPLINE_SURFACE(((1.,1.),(0.948102323621204,0.987087872581763),
(0.948102323621204,0.987087872581763),(1.,1.)))
REPRESENTATION_ITEM('')
SURFACE()
);
#3951=(
BOUNDED_SURFACE()
B_SPLINE_SURFACE(3,2,((#255695,#255696,#255697),(#255698,#255699,#255700),
(#255701,#255702,#255703),(#255704,#255705,#255706)),.UNSPECIFIED.,.F.,
 .F.,.F.)
B_SPLINE_SURFACE_WITH_KNOTS((4,4),(3,3),(-3.46944695195361E-18,0.00108749691872869),
(0.827141149879304,1.),.UNSPECIFIED.)
GEOMETRIC_REPRESENTATION_ITEM()
RATIONAL_B_SPLINE_SURFACE(((0.969924731391313,0.981819748290195,1.),(0.969924599712626,
0.981819668691515,1.),(0.969814841303219,0.981753320638693,1.),(0.969600878752829,
0.981623982042481,1.)))
REPRESENTATION_ITEM('')
SURFACE()
);
#3952=(
BOUNDED_SURFACE()
B_SPLINE_SURFACE(3,2,((#255790,#255791,#255792),(#255793,#255794,#255795),
(#255796,#255797,#255798),(#255799,#255800,#255801)),.UNSPECIFIED.,.F.,
 .F.,.F.)
B_SPLINE_SURFACE_WITH_KNOTS((4,4),(3,3),(0.,0.00108749691872869),(0.,0.172858850120678),
 .UNSPECIFIED.)
GEOMETRIC_REPRESENTATION_ITEM()
RATIONAL_B_SPLINE_SURFACE(((1.,0.981819748290197,0.969924731391315),(1.,
0.981819668691517,0.969924599712628),(1.,0.981753320638695,0.969814841303222),
(1.,0.981623982042483,0.969600878752832)))
REPRESENTATION_ITEM('')
SURFACE()
);
#3953=(
BOUNDED_SURFACE()
B_SPLINE_SURFACE(3,2,((#255884,#255885,#255886),(#255887,#255888,#255889),
(#255890,#255891,#255892),(#255893,#255894,#255895)),.UNSPECIFIED.,.F.,
 .F.,.F.)
B_SPLINE_SURFACE_WITH_KNOTS((4,4),(3,3),(0.,0.00108749691872869),(0.827141149879317,
1.),.UNSPECIFIED.)
GEOMETRIC_REPRESENTATION_ITEM()
RATIONAL_B_SPLINE_SURFACE(((0.969924731391315,0.981819748290196,1.),(0.969924599712627,
0.981819668691516,1.),(0.969814841303221,0.981753320638695,1.),(0.969600878752831,
0.981623982042482,1.)))
REPRESENTATION_ITEM('')
SURFACE()
);
#3954=(
BOUNDED_SURFACE()
B_SPLINE_SURFACE(3,2,((#255942,#255943,#255944),(#255945,#255946,#255947),
(#255948,#255949,#255950),(#255951,#255952,#255953)),.UNSPECIFIED.,.F.,
 .F.,.F.)
B_SPLINE_SURFACE_WITH_KNOTS((4,4),(3,3),(-3.46944695195361E-18,0.0010874969187287),
(0.,0.172858850120678),.UNSPECIFIED.)
GEOMETRIC_REPRESENTATION_ITEM()
RATIONAL_B_SPLINE_SURFACE(((1.,0.981819748290197,0.969924731391316),(1.,
0.981819668691517,0.969924599712629),(1.,0.981753320638695,0.969814841303222),
(1.,0.981623982042483,0.969600878752832)))
REPRESENTATION_ITEM('')
SURFACE()
);
#3955=(
BOUNDED_SURFACE()
B_SPLINE_SURFACE(3,2,((#256036,#256037,#256038),(#256039,#256040,#256041),
(#256042,#256043,#256044),(#256045,#256046,#256047)),.UNSPECIFIED.,.F.,
 .F.,.F.)
B_SPLINE_SURFACE_WITH_KNOTS((4,4),(3,3),(0.,0.00108749691872869),(0.82714114987934,
1.),.UNSPECIFIED.)
GEOMETRIC_REPRESENTATION_ITEM()
RATIONAL_B_SPLINE_SURFACE(((0.969924731391318,0.981819748290198,1.),(0.969924599712631,
0.981819668691519,1.),(0.969814841303224,0.981753320638697,1.),(0.969600878752834,
0.981623982042484,1.)))
REPRESENTATION_ITEM('')
SURFACE()
);
#3956=(
BOUNDED_SURFACE()
B_SPLINE_SURFACE(3,2,((#256130,#256131,#256132),(#256133,#256134,#256135),
(#256136,#256137,#256138),(#256139,#256140,#256141)),.UNSPECIFIED.,.F.,
 .F.,.F.)
B_SPLINE_SURFACE_WITH_KNOTS((4,4),(3,3),(-3.03576608295941E-18,0.00108749691872869),
(0.,0.172858850120729),.UNSPECIFIED.)
GEOMETRIC_REPRESENTATION_ITEM()
RATIONAL_B_SPLINE_SURFACE(((1.,0.981819748290191,0.969924731391308),(1.,
0.981819668691511,0.969924599712621),(1.,0.98175332063869,0.969814841303215),
(1.,0.981623982042477,0.969600878752825)))
REPRESENTATION_ITEM('')
SURFACE()
);
#3957=(
BOUNDED_SURFACE()
B_SPLINE_SURFACE(3,2,((#256154,#256155,#256156),(#256157,#256158,#256159),
(#256160,#256161,#256162),(#256163,#256164,#256165)),.UNSPECIFIED.,.F.,
 .F.,.F.)
B_SPLINE_SURFACE_WITH_KNOTS((4,4),(3,3),(0.,0.0010874969187287),(0.,0.172858850120729),
 .UNSPECIFIED.)
GEOMETRIC_REPRESENTATION_ITEM()
RATIONAL_B_SPLINE_SURFACE(((1.,0.981819748290191,0.969924731391308),(1.,
0.981819668691512,0.969924599712622),(1.,0.98175332063869,0.969814841303215),
(1.,0.981623982042477,0.969600878752825)))
REPRESENTATION_ITEM('')
SURFACE()
);
#3958=(
BOUNDED_SURFACE()
B_SPLINE_SURFACE(3,2,((#256178,#256179,#256180),(#256181,#256182,#256183),
(#256184,#256185,#256186),(#256187,#256188,#256189)),.UNSPECIFIED.,.F.,
 .F.,.F.)
B_SPLINE_SURFACE_WITH_KNOTS((4,4),(3,3),(0.,0.00108749691872868),(0.827141149879317,
1.),.UNSPECIFIED.)
GEOMETRIC_REPRESENTATION_ITEM()
RATIONAL_B_SPLINE_SURFACE(((0.969924731391315,0.981819748290196,1.),(0.969924599712628,
0.981819668691516,1.),(0.969814841303221,0.981753320638694,1.),(0.969600878752831,
0.981623982042482,1.)))
REPRESENTATION_ITEM('')
SURFACE()
);
#3959=(
BOUNDED_SURFACE()
B_SPLINE_SURFACE(2,2,((#256202,#256203,#256204),(#256205,#256206,#256207),
(#256208,#256209,#256210)),.UNSPECIFIED.,.F.,.F.,.F.)
B_SPLINE_SURFACE_WITH_KNOTS((3,3),(3,3),(-1.5707963267949,0.),(0.959931088596877,
1.88544105556098),.UNSPECIFIED.)
GEOMETRIC_REPRESENTATION_ITEM()
RATIONAL_B_SPLINE_SURFACE(((1.,0.894826028883615,1.),(0.707106781186545,
0.632737553005832,0.707106781186545),(1.,0.894826028883615,1.)))
REPRESENTATION_ITEM('')
SURFACE()
);
#3960=(
BOUNDED_SURFACE()
B_SPLINE_SURFACE(2,2,((#256219,#256220,#256221),(#256222,#256223,#256224),
(#256225,#256226,#256227)),.UNSPECIFIED.,.F.,.F.,.F.)
B_SPLINE_SURFACE_WITH_KNOTS((3,3),(3,3),(-1.5707963267949,0.),(1.25615159802882,
2.18166156499291),.UNSPECIFIED.)
GEOMETRIC_REPRESENTATION_ITEM()
RATIONAL_B_SPLINE_SURFACE(((1.,0.894826028883616,1.),(0.707106781186542,
0.632737553005829,0.707106781186542),(1.,0.894826028883616,1.)))
REPRESENTATION_ITEM('')
SURFACE()
);
#3961=(
BOUNDED_SURFACE()
B_SPLINE_SURFACE(3,2,((#256229,#256230,#256231),(#256232,#256233,#256234),
(#256235,#256236,#256237),(#256238,#256239,#256240),(#256241,#256242,#256243),
(#256244,#256245,#256246),(#256247,#256248,#256249),(#256250,#256251,#256252),
(#256253,#256254,#256255),(#256256,#256257,#256258),(#256259,#256260,#256261),
(#256262,#256263,#256264),(#256265,#256266,#256267),(#256268,#256269,#256270)),
 .UNSPECIFIED.,.F.,.F.,.F.)
B_SPLINE_SURFACE_WITH_KNOTS((4,2,2,2,2,2,4),(3,3),(0.00306933855977502,
0.00495218666169259,0.00683503476361015,0.00871788286552771,0.0106007309674453,
0.0143664271712804,0.0181321233751155),(0.,1.),.UNSPECIFIED.)
GEOMETRIC_REPRESENTATION_ITEM()
RATIONAL_B_SPLINE_SURFACE(((1.,0.707106781186548,1.),(1.,0.733011584422493,
1.),(1.,0.756757437792392,1.),(1.,0.800574796194754,1.),(1.,0.820645929370482,
1.),(1.,0.857475616581832,1.),(1.,0.874266151416803,1.),(1.,0.904559499542173,
1.),(1.,0.917975383131884,1.),(1.,0.953491353960086,1.),(1.,0.970901198269013,
1.),(1.,0.994190014771706,1.),(1.,1.00000947743974,1.),(1.,1.,1.)))
REPRESENTATION_ITEM('')
SURFACE()
);
#3962=(
BOUNDED_SURFACE()
B_SPLINE_SURFACE(3,2,((#256374,#256375,#256376),(#256377,#256378,#256379),
(#256380,#256381,#256382),(#256383,#256384,#256385),(#256386,#256387,#256388),
(#256389,#256390,#256391),(#256392,#256393,#256394),(#256395,#256396,#256397),
(#256398,#256399,#256400),(#256401,#256402,#256403),(#256404,#256405,#256406),
(#256407,#256408,#256409),(#256410,#256411,#256412),(#256413,#256414,#256415)),
 .UNSPECIFIED.,.F.,.F.,.F.)
B_SPLINE_SURFACE_WITH_KNOTS((4,2,2,2,2,2,4),(3,3),(0.00306933855977502,
0.00495218666169259,0.00683503476361015,0.00871788286552771,0.0106007309674453,
0.0143664271712804,0.0181321233751155),(0.,1.),.UNSPECIFIED.)
GEOMETRIC_REPRESENTATION_ITEM()
RATIONAL_B_SPLINE_SURFACE(((1.,0.707106781186548,1.),(1.,0.733011584422493,
1.),(1.,0.756757437792392,1.),(1.,0.800574796194754,1.),(1.,0.820645929370482,
1.),(1.,0.857475616581832,1.),(1.,0.874266151416803,1.),(1.,0.904559499542173,
1.),(1.,0.917975383131884,1.),(1.,0.953491353960086,1.),(1.,0.970901198269013,
1.),(1.,0.994190014771706,1.),(1.,1.00000947743974,1.),(1.,1.,1.)))
REPRESENTATION_ITEM('')
SURFACE()
);
#3963=(
BOUNDED_SURFACE()
B_SPLINE_SURFACE(3,2,((#256420,#256421,#256422),(#256423,#256424,#256425),
(#256426,#256427,#256428),(#256429,#256430,#256431),(#256432,#256433,#256434),
(#256435,#256436,#256437),(#256438,#256439,#256440),(#256441,#256442,#256443),
(#256444,#256445,#256446),(#256447,#256448,#256449),(#256450,#256451,#256452),
(#256453,#256454,#256455),(#256456,#256457,#256458),(#256459,#256460,#256461)),
 .UNSPECIFIED.,.F.,.F.,.F.)
B_SPLINE_SURFACE_WITH_KNOTS((4,2,2,2,2,2,4),(3,3),(0.003069338559775,0.00495218666169257,
0.00683503476361014,0.00871788286552772,0.0106007309674453,0.0143664271712804,
0.0181321233751156),(0.,1.),.UNSPECIFIED.)
GEOMETRIC_REPRESENTATION_ITEM()
RATIONAL_B_SPLINE_SURFACE(((1.,0.70710678118655,1.),(1.,0.73301158442153,
1.),(1.,0.756757437793674,1.),(1.,0.800574796193468,1.),(1.,0.82064592936982,
1.),(1.,0.85747561658249,1.),(1.,0.874266151415543,1.),(1.,0.904559499543433,
1.),(1.,0.917975383132164,1.),(1.,0.953491353959532,1.),(1.,0.970901198269014,
1.),(1.,0.994190014771708,1.),(1.,1.00000947743974,1.),(1.,1.,1.)))
REPRESENTATION_ITEM('')
SURFACE()
);
#3964=(
BOUNDED_SURFACE()
B_SPLINE_SURFACE(3,2,((#256565,#256566,#256567),(#256568,#256569,#256570),
(#256571,#256572,#256573),(#256574,#256575,#256576),(#256577,#256578,#256579),
(#256580,#256581,#256582),(#256583,#256584,#256585),(#256586,#256587,#256588),
(#256589,#256590,#256591),(#256592,#256593,#256594),(#256595,#256596,#256597),
(#256598,#256599,#256600),(#256601,#256602,#256603),(#256604,#256605,#256606)),
 .UNSPECIFIED.,.F.,.F.,.F.)
B_SPLINE_SURFACE_WITH_KNOTS((4,2,2,2,2,2,4),(3,3),(0.003069338559775,0.00495218666169257,
0.00683503476361014,0.00871788286552772,0.0106007309674453,0.0143664271712804,
0.0181321233751156),(0.,1.),.UNSPECIFIED.)
GEOMETRIC_REPRESENTATION_ITEM()
RATIONAL_B_SPLINE_SURFACE(((1.,0.70710678118655,1.),(1.,0.73301158442153,
1.),(1.,0.756757437793674,1.),(1.,0.800574796193468,1.),(1.,0.82064592936982,
1.),(1.,0.85747561658249,1.),(1.,0.874266151415543,1.),(1.,0.904559499543433,
1.),(1.,0.917975383132164,1.),(1.,0.953491353959532,1.),(1.,0.970901198269014,
1.),(1.,0.994190014771708,1.),(1.,1.00000947743974,1.),(1.,1.,1.)))
REPRESENTATION_ITEM('')
SURFACE()
);
#3965=(
BOUNDED_SURFACE()
B_SPLINE_SURFACE(3,2,((#256612,#256613,#256614),(#256615,#256616,#256617),
(#256618,#256619,#256620),(#256621,#256622,#256623),(#256624,#256625,#256626),
(#256627,#256628,#256629),(#256630,#256631,#256632),(#256633,#256634,#256635),
(#256636,#256637,#256638),(#256639,#256640,#256641),(#256642,#256643,#256644),
(#256645,#256646,#256647),(#256648,#256649,#256650),(#256651,#256652,#256653)),
 .UNSPECIFIED.,.F.,.F.,.F.)
B_SPLINE_SURFACE_WITH_KNOTS((4,2,2,2,2,2,4),(3,3),(0.00306933855977502,
0.00495218666169259,0.00683503476361016,0.00871788286552773,0.0106007309674453,
0.0143664271712804,0.0181321233751156),(0.,1.),.UNSPECIFIED.)
GEOMETRIC_REPRESENTATION_ITEM()
RATIONAL_B_SPLINE_SURFACE(((1.,0.70710678118655,1.),(1.,0.73301158442153,
1.),(1.,0.756757437793674,1.),(1.,0.800574796193468,1.),(1.,0.820645929369924,
1.),(1.,0.857475616582386,1.),(1.,0.874266151416033,1.),(1.,0.904559499542943,
1.),(1.,0.917975383132164,1.),(1.,0.953491353959532,1.),(1.,0.970901198268875,
1.),(1.,0.994190014771847,1.),(1.,1.00000947743964,1.),(1.,1.,1.)))
REPRESENTATION_ITEM('')
SURFACE()
);
#3966=(
BOUNDED_SURFACE()
B_SPLINE_SURFACE(3,2,((#256757,#256758,#256759),(#256760,#256761,#256762),
(#256763,#256764,#256765),(#256766,#256767,#256768),(#256769,#256770,#256771),
(#256772,#256773,#256774),(#256775,#256776,#256777),(#256778,#256779,#256780),
(#256781,#256782,#256783),(#256784,#256785,#256786),(#256787,#256788,#256789),
(#256790,#256791,#256792),(#256793,#256794,#256795),(#256796,#256797,#256798)),
 .UNSPECIFIED.,.F.,.F.,.F.)
B_SPLINE_SURFACE_WITH_KNOTS((4,2,2,2,2,2,4),(3,3),(0.00306933855977502,
0.00495218666169259,0.00683503476361016,0.00871788286552773,0.0106007309674453,
0.0143664271712804,0.0181321233751156),(0.,1.),.UNSPECIFIED.)
GEOMETRIC_REPRESENTATION_ITEM()
RATIONAL_B_SPLINE_SURFACE(((1.,0.70710678118655,1.),(1.,0.73301158442153,
1.),(1.,0.756757437793674,1.),(1.,0.800574796193468,1.),(1.,0.820645929369924,
1.),(1.,0.857475616582386,1.),(1.,0.874266151416033,1.),(1.,0.904559499542943,
1.),(1.,0.917975383132164,1.),(1.,0.953491353959532,1.),(1.,0.970901198268875,
1.),(1.,0.994190014771847,1.),(1.,1.00000947743964,1.),(1.,1.,1.)))
REPRESENTATION_ITEM('')
SURFACE()
);
#3967=(
BOUNDED_SURFACE()
B_SPLINE_SURFACE(3,2,((#256801,#256802,#256803),(#256804,#256805,#256806),
(#256807,#256808,#256809),(#256810,#256811,#256812),(#256813,#256814,#256815),
(#256816,#256817,#256818),(#256819,#256820,#256821),(#256822,#256823,#256824),
(#256825,#256826,#256827),(#256828,#256829,#256830),(#256831,#256832,#256833),
(#256834,#256835,#256836),(#256837,#256838,#256839),(#256840,#256841,#256842)),
 .UNSPECIFIED.,.F.,.F.,.F.)
B_SPLINE_SURFACE_WITH_KNOTS((4,2,2,2,2,2,4),(3,3),(0.0165800150464154,0.0218443656748581,
0.0271029672948129,0.0376201705347225,0.048137373774632,0.0533959753945868,
0.0586603260230295),(0.,1.00000574900849),.UNSPECIFIED.)
GEOMETRIC_REPRESENTATION_ITEM()
RATIONAL_B_SPLINE_SURFACE(((1.,0.746871247280354,1.0000029104787),(1.,0.745462351055241,
1.00000292667821),(1.,0.744212008056876,1.00000294105467),(1.,0.742063457964921,
1.00000296575874),(1.,0.741161631619667,1.00000297612795),(1.,0.738982445187317,
1.00000300118428),(1.,0.738228768574483,1.00000300985006),(1.,0.738231075589957,
1.00000300982354),(1.,0.738986907486423,1.00000300113297),(1.,0.741166319133875,
1.00000297607406),(1.,0.742067724836351,1.00000296570968),(1.,0.744213991604145,
1.00000294103187),(1.,0.745461255089228,1.00000292669081),(1.,0.746871250867751,
1.00000291047865)))
REPRESENTATION_ITEM('')
SURFACE()
);
#3968=(
BOUNDED_SURFACE()
B_SPLINE_SURFACE(3,2,((#257652,#257653,#257654),(#257655,#257656,#257657),
(#257658,#257659,#257660),(#257661,#257662,#257663),(#257664,#257665,#257666),
(#257667,#257668,#257669),(#257670,#257671,#257672),(#257673,#257674,#257675),
(#257676,#257677,#257678),(#257679,#257680,#257681),(#257682,#257683,#257684),
(#257685,#257686,#257687),(#257688,#257689,#257690),(#257691,#257692,#257693),
(#257694,#257695,#257696),(#257697,#257698,#257699),(#257700,#257701,#257702),
(#257703,#257704,#257705),(#257706,#257707,#257708),(#257709,#257710,#257711),
(#257712,#257713,#257714),(#257715,#257716,#257717)),.UNSPECIFIED.,.F.,
 .F.,.F.)
B_SPLINE_SURFACE_WITH_KNOTS((4,2,2,2,2,2,2,2,2,2,4),(3,3),(0.00948259018043931,
0.0103154262700519,0.0111482623596645,0.0119810984492771,0.0123975164940833,
0.0128139345388896,0.0136467706285022,0.0144796067181148,0.0148960247629211,
0.0153124428077274,0.01614527889734),(0.,1.),.UNSPECIFIED.)
GEOMETRIC_REPRESENTATION_ITEM()
RATIONAL_B_SPLINE_SURFACE(((1.,0.748955720789,1.),(1.,0.760172974879871,
1.),(1.,0.771047258289343,1.),(1.,0.792164805631483,1.),(1.,0.80250638759394,
1.),(1.,0.821938683277389,1.),(1.,0.831055189778017,1.),(1.,0.843821930267136,
1.),(1.,0.847925078305043,1.),(1.,0.855808932317141,1.),(1.,0.859614300419405,
1.),(1.,0.870277583221261,1.),(1.,0.876401549840479,1.),(1.,0.886526706071859,
1.),(1.,0.890548210266271,1.),(1.,0.894400461302912,1.),(1.,0.895338782452369,
1.),(1.,0.896497135067161,1.),(1.,0.896712673869112,1.),(1.,0.89622893258817,
1.),(1.,0.894438559265301,1.),(1.,0.891217425172869,1.)))
REPRESENTATION_ITEM('')
SURFACE()
);
#3969=(
BOUNDED_SURFACE()
B_SPLINE_SURFACE(3,2,((#257892,#257893,#257894),(#257895,#257896,#257897),
(#257898,#257899,#257900),(#257901,#257902,#257903),(#257904,#257905,#257906),
(#257907,#257908,#257909),(#257910,#257911,#257912),(#257913,#257914,#257915),
(#257916,#257917,#257918),(#257919,#257920,#257921),(#257922,#257923,#257924),
(#257925,#257926,#257927),(#257928,#257929,#257930),(#257931,#257932,#257933),
(#257934,#257935,#257936),(#257937,#257938,#257939),(#257940,#257941,#257942),
(#257943,#257944,#257945),(#257946,#257947,#257948),(#257949,#257950,#257951)),
 .UNSPECIFIED.,.F.,.F.,.F.)
B_SPLINE_SURFACE_WITH_KNOTS((4,2,2,2,2,2,2,2,2,4),(3,3),(0.0112764198461947,
0.0121119087584978,0.0125296532146494,0.012947397670801,0.0137828865831041,
0.0146183754954072,0.0154538644077104,0.0162893533200135,0.0171248422323166,
0.0179603311446198),(0.,1.),.UNSPECIFIED.)
GEOMETRIC_REPRESENTATION_ITEM()
RATIONAL_B_SPLINE_SURFACE(((1.,0.89121897909325,1.),(1.,0.894429433227244,
1.),(1.,0.896207982264178,1.),(1.,0.896714045563393,1.),(1.,0.896515267970691,
1.),(1.,0.895381325101059,1.),(1.,0.894455556169836,1.),(1.,0.890656783919795,
1.),(1.,0.886687750370936,1.),(1.,0.876609320012727,1.),(1.,0.870508986223097,
1.),(1.,0.856349909354098,1.),(1.,0.84841920915651,1.),(1.,0.831316008677178,
1.),(1.,0.822011223917002,1.),(1.,0.8025589034124,1.),(1.,0.792407582621121,
1.),(1.,0.771230982137234,1.),(1.,0.760139004795012,1.),(1.,0.748955720789,
1.)))
REPRESENTATION_ITEM('')
SURFACE()
);
#3970=(
BOUNDED_SURFACE()
B_SPLINE_SURFACE(3,2,((#258120,#258121,#258122),(#258123,#258124,#258125),
(#258126,#258127,#258128),(#258129,#258130,#258131),(#258132,#258133,#258134),
(#258135,#258136,#258137),(#258138,#258139,#258140),(#258141,#258142,#258143),
(#258144,#258145,#258146),(#258147,#258148,#258149),(#258150,#258151,#258152),
(#258153,#258154,#258155),(#258156,#258157,#258158),(#258159,#258160,#258161),
(#258162,#258163,#258164),(#258165,#258166,#258167),(#258168,#258169,#258170),
(#258171,#258172,#258173),(#258174,#258175,#258176),(#258177,#258178,#258179),
(#258180,#258181,#258182),(#258183,#258184,#258185)),.UNSPECIFIED.,.F.,
 .F.,.F.)
B_SPLINE_SURFACE_WITH_KNOTS((4,2,2,2,2,2,2,2,2,2,4),(3,3),(0.0094825901804395,
0.0103154262700525,0.0111482623596655,0.0119810984492784,0.0123975164940849,
0.0128139345388914,0.0136467706285044,0.0144796067181174,0.0148960247629239,
0.0153124428077303,0.0161452788973433),(0.,1.),.UNSPECIFIED.)
GEOMETRIC_REPRESENTATION_ITEM()
RATIONAL_B_SPLINE_SURFACE(((1.,0.748955720789002,1.),(1.,0.76017297487987,
1.),(1.,0.771047258289371,1.),(1.,0.792164805631491,1.),(1.,0.802506387593797,
1.),(1.,0.821938683277595,1.),(1.,0.83105518977779,1.),(1.,0.843821930267307,
1.),(1.,0.847925078305022,1.),(1.,0.855808932317248,1.),(1.,0.859614300419415,
1.),(1.,0.87027758322137,1.),(1.,0.876401549840654,1.),(1.,0.88652670607176,
1.),(1.,0.890548210266293,1.),(1.,0.894400461302936,1.),(1.,0.895338782452428,
1.),(1.,0.896497135067126,1.),(1.,0.896712673869015,1.),(1.,0.896228932588355,
1.),(1.,0.894438559265128,1.),(1.,0.891217425172832,1.)))
REPRESENTATION_ITEM('')
SURFACE()
);
#3971=(
BOUNDED_SURFACE()
B_SPLINE_SURFACE(3,2,((#258360,#258361,#258362),(#258363,#258364,#258365),
(#258366,#258367,#258368),(#258369,#258370,#258371),(#258372,#258373,#258374),
(#258375,#258376,#258377),(#258378,#258379,#258380),(#258381,#258382,#258383),
(#258384,#258385,#258386),(#258387,#258388,#258389),(#258390,#258391,#258392),
(#258393,#258394,#258395),(#258396,#258397,#258398),(#258399,#258400,#258401),
(#258402,#258403,#258404),(#258405,#258406,#258407),(#258408,#258409,#258410),
(#258411,#258412,#258413),(#258414,#258415,#258416),(#258417,#258418,#258419)),
 .UNSPECIFIED.,.F.,.F.,.F.)
B_SPLINE_SURFACE_WITH_KNOTS((4,2,2,2,2,2,2,2,2,4),(3,3),(0.0112764198461948,
0.0121119087584979,0.0125296532146495,0.0129473976708011,0.0137828865831043,
0.0146183754954074,0.0154538644077106,0.0162893533200137,0.0171248422323169,
0.0179603311446201),(0.,1.),.UNSPECIFIED.)
GEOMETRIC_REPRESENTATION_ITEM()
RATIONAL_B_SPLINE_SURFACE(((1.,0.891218979093247,1.),(1.,0.89442943322708,
1.),(1.,0.896207982264393,1.),(1.,0.896714045563283,1.),(1.,0.896515267970747,
1.),(1.,0.895381325101006,1.),(1.,0.894455556169837,1.),(1.,0.890656783919796,
1.),(1.,0.886687750370708,1.),(1.,0.876609320012963,1.),(1.,0.870508986222868,
1.),(1.,0.856349909354336,1.),(1.,0.848419209156267,1.),(1.,0.831316008677429,
1.),(1.,0.822011223916974,1.),(1.,0.802558903412434,1.),(1.,0.792407582620859,
1.),(1.,0.771230982137498,1.),(1.,0.760139004794817,1.),(1.,0.748955720788999,
1.)))
REPRESENTATION_ITEM('')
SURFACE()
);
#3972=(
BOUNDED_SURFACE()
B_SPLINE_SURFACE(3,2,((#258588,#258589,#258590),(#258591,#258592,#258593),
(#258594,#258595,#258596),(#258597,#258598,#258599),(#258600,#258601,#258602),
(#258603,#258604,#258605),(#258606,#258607,#258608),(#258609,#258610,#258611),
(#258612,#258613,#258614),(#258615,#258616,#258617),(#258618,#258619,#258620),
(#258621,#258622,#258623),(#258624,#258625,#258626),(#258627,#258628,#258629),
(#258630,#258631,#258632),(#258633,#258634,#258635),(#258636,#258637,#258638),
(#258639,#258640,#258641),(#258642,#258643,#258644),(#258645,#258646,#258647),
(#258648,#258649,#258650),(#258651,#258652,#258653)),.UNSPECIFIED.,.F.,
 .F.,.F.)
B_SPLINE_SURFACE_WITH_KNOTS((4,2,2,2,2,2,2,2,2,2,4),(3,3),(0.00948259018043928,
0.0103154262700518,0.0111482623596644,0.011981098449277,0.0123975164940833,
0.0128139345388895,0.0136467706285021,0.0144796067181147,0.0148960247629209,
0.0153124428077272,0.0161452788973398),(0.,1.),.UNSPECIFIED.)
GEOMETRIC_REPRESENTATION_ITEM()
RATIONAL_B_SPLINE_SURFACE(((1.,0.748955720789,1.),(1.,0.760172974879684,
1.),(1.,0.771047258289592,1.),(1.,0.792164805631237,1.),(1.,0.8025063875938,
1.),(1.,0.821938683277527,1.),(1.,0.831055189777864,1.),(1.,0.843821930267213,
1.),(1.,0.847925078305238,1.),(1.,0.855808932316948,1.),(1.,0.859614300419269,
1.),(1.,0.870277583221523,1.),(1.,0.876401549840585,1.),(1.,0.886526706071749,
1.),(1.,0.890548210266254,1.),(1.,0.894400461302918,1.),(1.,0.895338782452494,
1.),(1.,0.896497135067036,1.),(1.,0.896712673869119,1.),(1.,0.896228932588154,
1.),(1.,0.894438559265315,1.),(1.,0.89121742517287,1.)))
REPRESENTATION_ITEM('')
SURFACE()
);
#3973=(
BOUNDED_SURFACE()
B_SPLINE_SURFACE(3,2,((#258828,#258829,#258830),(#258831,#258832,#258833),
(#258834,#258835,#258836),(#258837,#258838,#258839),(#258840,#258841,#258842),
(#258843,#258844,#258845),(#258846,#258847,#258848),(#258849,#258850,#258851),
(#258852,#258853,#258854),(#258855,#258856,#258857),(#258858,#258859,#258860),
(#258861,#258862,#258863),(#258864,#258865,#258866),(#258867,#258868,#258869),
(#258870,#258871,#258872),(#258873,#258874,#258875),(#258876,#258877,#258878),
(#258879,#258880,#258881)),.UNSPECIFIED.,.F.,.F.,.F.)
B_SPLINE_SURFACE_WITH_KNOTS((4,2,2,2,2,2,2,2,4),(3,3),(0.0113523220585582,
0.012178323194316,0.0125913237621948,0.0130043243300737,0.0138303254658314,
0.0146563266015892,0.0154823277373469,0.0163083288731046,0.0179603311446201),
(0.,1.),.UNSPECIFIED.)
GEOMETRIC_REPRESENTATION_ITEM()
RATIONAL_B_SPLINE_SURFACE(((1.,0.892059672490622,1.),(1.,0.89497186029643,
1.),(1.,0.896493669878046,1.),(1.,0.89665049960315,1.),(1.,0.896338830961171,
1.),(1.,0.895008636648382,1.),(1.,0.893996388994617,1.),(1.,0.889965092157251,
1.),(1.,0.885881976568346,1.),(1.,0.875677600351648,1.),(1.,0.869546831587427,
1.),(1.,0.855370301029908,1.),(1.,0.847491252571126,1.),(1.,0.83049125023834,
1.),(1.,0.82125667883682,1.),(1.,0.792351743707096,1.),(1.,0.771269968248487,
1.),(1.,0.748955720788999,1.)))
REPRESENTATION_ITEM('')
SURFACE()
);
#3974=(
BOUNDED_SURFACE()
B_SPLINE_SURFACE(3,2,((#259007,#259008,#259009),(#259010,#259011,#259012),
(#259013,#259014,#259015),(#259016,#259017,#259018),(#259019,#259020,#259021),
(#259022,#259023,#259024),(#259025,#259026,#259027),(#259028,#259029,#259030),
(#259031,#259032,#259033),(#259034,#259035,#259036),(#259037,#259038,#259039),
(#259040,#259041,#259042),(#259043,#259044,#259045),(#259046,#259047,#259048),
(#259049,#259050,#259051),(#259052,#259053,#259054),(#259055,#259056,#259057),
(#259058,#259059,#259060),(#259061,#259062,#259063),(#259064,#259065,#259066)),
 .UNSPECIFIED.,.F.,.F.,.F.)
B_SPLINE_SURFACE_WITH_KNOTS((4,2,2,2,2,2,2,2,2,4),(3,3),(0.0112764198461918,
0.0121119087584954,0.0125296532146471,0.0129473976707989,0.0137828865831024,
0.0146183754954059,0.0154538644077094,0.016289353320013,0.0171248422323165,
0.01796033114462),(0.,1.),.UNSPECIFIED.)
GEOMETRIC_REPRESENTATION_ITEM()
RATIONAL_B_SPLINE_SURFACE(((1.,0.891218979093214,1.),(1.,0.894429433227121,
1.),(1.,0.896207982264297,1.),(1.,0.896714045563326,1.),(1.,0.896515267970734,
1.),(1.,0.895381325101037,1.),(1.,0.894455556169857,1.),(1.,0.890656783919815,
1.),(1.,0.88668775037085,1.),(1.,0.876609320012884,1.),(1.,0.870508986223,
1.),(1.,0.856349909354275,1.),(1.,0.848419209156365,1.),(1.,0.831316008677397,
1.),(1.,0.822011223917237,1.),(1.,0.802558903412222,1.),(1.,0.792407582620879,
1.),(1.,0.771230982137509,1.),(1.,0.760139004794819,1.),(1.,0.748955720789001,
1.)))
REPRESENTATION_ITEM('')
SURFACE()
);
#3975=(
BOUNDED_SURFACE()
B_SPLINE_SURFACE(3,2,((#259238,#259239,#259240),(#259241,#259242,#259243),
(#259244,#259245,#259246),(#259247,#259248,#259249),(#259250,#259251,#259252),
(#259253,#259254,#259255),(#259256,#259257,#259258),(#259259,#259260,#259261),
(#259262,#259263,#259264),(#259265,#259266,#259267),(#259268,#259269,#259270),
(#259271,#259272,#259273),(#259274,#259275,#259276),(#259277,#259278,#259279),
(#259280,#259281,#259282),(#259283,#259284,#259285),(#259286,#259287,#259288),
(#259289,#259290,#259291),(#259292,#259293,#259294),(#259295,#259296,#259297),
(#259298,#259299,#259300),(#259301,#259302,#259303)),.UNSPECIFIED.,.F.,
 .F.,.F.)
B_SPLINE_SURFACE_WITH_KNOTS((4,2,2,2,2,2,2,2,2,2,4),(3,3),(0.00948259018043951,
0.0103154262700521,0.0111482623596647,0.0119810984492773,0.0123975164940836,
0.0128139345388899,0.0136467706285025,0.0144796067181151,0.0148960247629214,
0.0153124428077277,0.0161452788973402),(0.,1.),.UNSPECIFIED.)
GEOMETRIC_REPRESENTATION_ITEM()
RATIONAL_B_SPLINE_SURFACE(((1.,0.748955720789002,1.),(1.,0.760172974879873,
1.),(1.,0.771047258289347,1.),(1.,0.792164805631487,1.),(1.,0.802506387594021,
1.),(1.,0.821938683277315,1.),(1.,0.831055189777944,1.),(1.,0.843821930267178,
1.),(1.,0.847925078304869,1.),(1.,0.855808932317324,1.),(1.,0.859614300419331,
1.),(1.,0.870277583221421,1.),(1.,0.87640154984062,1.),(1.,0.886526706071721,
1.),(1.,0.890548210266257,1.),(1.,0.894400461302922,1.),(1.,0.895338782452309,
1.),(1.,0.896497135067225,1.),(1.,0.896712673869011,1.),(1.,0.896228932588374,
1.),(1.,0.894438559265147,1.),(1.,0.891217425172868,1.)))
REPRESENTATION_ITEM('')
SURFACE()
);
#3976=(
BOUNDED_SURFACE()
B_SPLINE_SURFACE(3,2,((#259475,#259476,#259477),(#259478,#259479,#259480),
(#259481,#259482,#259483),(#259484,#259485,#259486)),.UNSPECIFIED.,.F.,
 .F.,.F.)
B_SPLINE_SURFACE_WITH_KNOTS((4,4),(3,3),(0.,0.0230962378966021),(0.,1.),
 .UNSPECIFIED.)
GEOMETRIC_REPRESENTATION_ITEM()
RATIONAL_B_SPLINE_SURFACE(((1.,0.75328262365528,1.),(1.,0.753799666532188,
1.),(1.,0.754334066265409,1.),(1.,0.754887701397112,1.)))
REPRESENTATION_ITEM('')
SURFACE()
);
#3977=(
BOUNDED_SURFACE()
B_SPLINE_SURFACE(3,2,((#259540,#259541,#259542),(#259543,#259544,#259545),
(#259546,#259547,#259548),(#259549,#259550,#259551)),.UNSPECIFIED.,.F.,
 .F.,.F.)
B_SPLINE_SURFACE_WITH_KNOTS((4,4),(3,3),(0.,0.000930412332424302),(0.,1.),
 .UNSPECIFIED.)
GEOMETRIC_REPRESENTATION_ITEM()
RATIONAL_B_SPLINE_SURFACE(((1.,0.753587188732319,1.),(1.,0.753587087859367,
1.),(1.,0.75348573487314,1.),(1.,0.75328262365528,1.)))
REPRESENTATION_ITEM('')
SURFACE()
);
#3978=(
BOUNDED_SURFACE()
B_SPLINE_SURFACE(3,2,((#259560,#259561,#259562),(#259563,#259564,#259565),
(#259566,#259567,#259568),(#259569,#259570,#259571)),.UNSPECIFIED.,.F.,
 .F.,.F.)
B_SPLINE_SURFACE_WITH_KNOTS((4,4),(3,3),(0.,0.023096237896602),(0.,1.),
 .UNSPECIFIED.)
GEOMETRIC_REPRESENTATION_ITEM()
RATIONAL_B_SPLINE_SURFACE(((1.,0.75328262365528,1.),(1.,0.753799666532188,
1.),(1.,0.75433406626541,1.),(1.,0.754887701397112,1.)))
REPRESENTATION_ITEM('')
SURFACE()
);
#3979=(
BOUNDED_SURFACE()
B_SPLINE_SURFACE(3,2,((#259613,#259614,#259615),(#259616,#259617,#259618),
(#259619,#259620,#259621),(#259622,#259623,#259624)),.UNSPECIFIED.,.F.,
 .F.,.F.)
B_SPLINE_SURFACE_WITH_KNOTS((4,4),(3,3),(-3.03576608295941E-18,0.000930412332424306),
(0.,1.),.UNSPECIFIED.)
GEOMETRIC_REPRESENTATION_ITEM()
RATIONAL_B_SPLINE_SURFACE(((1.,0.753587188732319,1.),(1.,0.753587087859366,
1.),(1.,0.75348573487314,1.),(1.,0.75328262365528,1.)))
REPRESENTATION_ITEM('')
SURFACE()
);
#3980=(
BOUNDED_SURFACE()
B_SPLINE_SURFACE(3,2,((#259633,#259634,#259635),(#259636,#259637,#259638),
(#259639,#259640,#259641),(#259642,#259643,#259644),(#259645,#259646,#259647),
(#259648,#259649,#259650)),.UNSPECIFIED.,.F.,.F.,.F.)
B_SPLINE_SURFACE_WITH_KNOTS((4,2,4),(3,3),(-1.65496705948116E-5,0.0175045710699778,
0.0350091421399555),(-1.65496705948116E-5,1.),.UNSPECIFIED.)
GEOMETRIC_REPRESENTATION_ITEM()
RATIONAL_B_SPLINE_SURFACE(((1.00000066361291,0.979950872403389,1.),(1.00000060946638,
0.981586752043857,1.),(1.00000054507474,0.983532157510661,1.),(1.00000038175755,
0.988466309672037,1.),(1.00000028087796,0.991514092184472,1.),(1.00000016544838,
0.995001460146994,1.)))
REPRESENTATION_ITEM('')
SURFACE()
);
#3981=(
BOUNDED_SURFACE()
B_SPLINE_SURFACE(3,2,((#259653,#259654,#259655),(#259656,#259657,#259658),
(#259659,#259660,#259661),(#259662,#259663,#259664),(#259665,#259666,#259667),
(#259668,#259669,#259670)),.UNSPECIFIED.,.F.,.F.,.F.)
B_SPLINE_SURFACE_WITH_KNOTS((4,2,4),(3,3),(-1.65496862290218E-5,0.0175045710699895,
0.0350091421399791),(0.,1.00001654968623),.UNSPECIFIED.)
GEOMETRIC_REPRESENTATION_ITEM()
RATIONAL_B_SPLINE_SURFACE(((1.,0.979950872398696,1.00000066361354),(1.,
0.981586752040342,1.00000060946695),(1.,0.98353215750788,1.00000054507525),
(1.,0.988466309672187,1.00000038175791),(1.,0.991514092184107,1.00000028087822),
(1.,0.99500146014693,1.00000016544853)))
REPRESENTATION_ITEM('')
SURFACE()
);
#3982=(
BOUNDED_SURFACE()
B_SPLINE_SURFACE(3,2,((#259673,#259674,#259675),(#259676,#259677,#259678),
(#259679,#259680,#259681),(#259682,#259683,#259684),(#259685,#259686,#259687),
(#259688,#259689,#259690),(#259691,#259692,#259693),(#259694,#259695,#259696),
(#259697,#259698,#259699),(#259700,#259701,#259702)),.UNSPECIFIED.,.F.,
 .F.,.F.)
B_SPLINE_SURFACE_WITH_KNOTS((4,2,2,2,4),(3,3),(0.0086793904370147,0.0137994096303372,
0.0163087030209128,0.0188179964114884,0.0289567865427477),(-0.000220356291476092,
1.),.UNSPECIFIED.)
GEOMETRIC_REPRESENTATION_ITEM()
RATIONAL_B_SPLINE_SURFACE(((1.0001233642456,0.720080046788299,0.999999999999999),
(1.00012059154998,0.726371438799624,1.),(1.00011860533177,0.73087827224561,
1.),(1.00011665984081,0.735292693407743,1.),(1.00011618394181,0.736372533239929,
1.),(1.00011554908712,0.737813051874643,1.),(1.00011539013292,0.738173727316974,
1.),(1.00011539009736,0.738173807996126,1.),(1.00011790792365,0.732460727893791,
1.),(1.00012336347158,0.720081803084609,1.)))
REPRESENTATION_ITEM('')
SURFACE()
);
#3983=(
BOUNDED_SURFACE()
B_SPLINE_SURFACE(3,2,((#259703,#259704,#259705),(#259706,#259707,#259708),
(#259709,#259710,#259711),(#259712,#259713,#259714)),.UNSPECIFIED.,.F.,
 .F.,.F.)
B_SPLINE_SURFACE_WITH_KNOTS((4,4),(3,3),(-1.0256276502154E-5,0.000591581032812799),
(0.,1.00225319390743),.UNSPECIFIED.)
GEOMETRIC_REPRESENTATION_ITEM()
RATIONAL_B_SPLINE_SURFACE(((1.,1.,1.),(1.,0.999985346901776,1.00000006603254),
(1.,0.99550874156864,1.00002023935227),(1.,0.988241468901958,1.00005298850126)))
REPRESENTATION_ITEM('')
SURFACE()
);
#3984=(
BOUNDED_SURFACE()
B_SPLINE_SURFACE(3,2,((#259725,#259726,#259727),(#259728,#259729,#259730),
(#259731,#259732,#259733),(#259734,#259735,#259736)),.UNSPECIFIED.,.F.,
 .F.,.F.)
B_SPLINE_SURFACE_WITH_KNOTS((4,4),(3,3),(-2.90836419617607E-14,0.000545703078886337),
(-0.00848691895860184,1.),.UNSPECIFIED.)
GEOMETRIC_REPRESENTATION_ITEM()
RATIONAL_B_SPLINE_SURFACE(((1.00000837657878,0.999506500603085,1.),(1.00000181717849,
0.999892942391636,1.),(1.00000000707574,0.999999583138454,1.),(1.,1.,1.)))
REPRESENTATION_ITEM('')
SURFACE()
);
#3985=(
BOUNDED_SURFACE()
B_SPLINE_SURFACE(3,2,((#259738,#259739,#259740),(#259741,#259742,#259743),
(#259744,#259745,#259746),(#259747,#259748,#259749),(#259750,#259751,#259752),
(#259753,#259754,#259755),(#259756,#259757,#259758),(#259759,#259760,#259761),
(#259762,#259763,#259764),(#259765,#259766,#259767),(#259768,#259769,#259770),
(#259771,#259772,#259773),(#259774,#259775,#259776),(#259777,#259778,#259779),
(#259780,#259781,#259782),(#259783,#259784,#259785),(#259786,#259787,#259788),
(#259789,#259790,#259791),(#259792,#259793,#259794),(#259795,#259796,#259797),
(#259798,#259799,#259800),(#259801,#259802,#259803),(#259804,#259805,#259806),
(#259807,#259808,#259809)),.UNSPECIFIED.,.F.,.F.,.F.)
B_SPLINE_SURFACE_WITH_KNOTS((4,2,2,2,2,2,2,2,2,2,2,4),(3,3),(0.00710973580532299,
0.00820484501164228,0.00898706587329885,0.00976928673495541,0.0101603971657837,
0.0103559523811978,0.0104537299889049,0.0104781743908317,0.0105026187927584,
0.0105270631946852,0.0105392853956486,0.0108643959412746),(-0.000692463643722109,
1.00461072647643),.UNSPECIFIED.)
GEOMETRIC_REPRESENTATION_ITEM()
RATIONAL_B_SPLINE_SURFACE(((1.00000418087808,0.996967228287315,1.00002794712048),
(1.00000539179128,0.996088842637076,1.00003604148165),(1.00000726417762,
0.994730630263104,1.00004855746652),(1.00001073944744,0.992209700500032,
1.00007178794164),(1.00001228661455,0.991087399257731,1.00008212999538),
(1.00001544659885,0.988795174797729,1.00010325294139),(1.00001711982762,
0.987581429549803,1.00011443765554),(1.00001894473692,0.986257656599376,
1.00012663627965),(1.00001951290412,0.985845513177767,1.00013043419883),
(1.00001922291158,0.98605587117993,1.00012849574088),(1.00001901775458,
0.986204690244211,1.00012712436687),(1.00001719907502,0.987523944194307,
1.00011496738554),(1.00001645641015,0.98806266667551,1.00011000303493),
(1.0000138946614,0.989920936399478,1.00009287900029),(1.00001328788623,
0.990361085704145,1.0000888230057),(1.00001167839794,0.991528594169834,
1.00007806436548),(1.00001068816558,0.992246899899225,1.00007144514759),
(1.00000775165148,0.99437702106797,1.00005181599031),(1.00000547142344,
0.996031078173962,1.00003657378364),(1.000002398545,0.998260116824386,1.00001603309756),
(1.00000153695282,0.998885108118202,1.00001027377617),(0.999987792404643,
1.00885528092366,0.999918398209191),(1.00027966865476,0.797130849193336,
1.00186944786376),(0.997855728441201,2.55543548703647,0.985666595749524)))
REPRESENTATION_ITEM('')
SURFACE()
);
#3986=(
BOUNDED_SURFACE()
B_SPLINE_SURFACE(3,2,((#259811,#259812,#259813),(#259814,#259815,#259816),
(#259817,#259818,#259819),(#259820,#259821,#259822)),.UNSPECIFIED.,.F.,
 .F.,.F.)
B_SPLINE_SURFACE_WITH_KNOTS((4,4),(3,3),(-2.85745148634754E-5,0.000314319663498228),
(0.,1.00095479621378),.UNSPECIFIED.)
GEOMETRIC_REPRESENTATION_ITEM()
RATIONAL_B_SPLINE_SURFACE(((1.,0.995946994781572,1.00000773958807),(1.,
0.996651841079251,1.00000639361892),(1.,0.997316919425854,1.00000512359035),
(1.,0.997737992799635,1.00000431951182)))
REPRESENTATION_ITEM('')
SURFACE()
);
#3987=(
BOUNDED_SURFACE()
B_SPLINE_SURFACE(3,2,((#259824,#259825,#259826),(#259827,#259828,#259829),
(#259830,#259831,#259832),(#259833,#259834,#259835)),.UNSPECIFIED.,.F.,
 .F.,.F.)
B_SPLINE_SURFACE_WITH_KNOTS((4,4),(3,3),(0.,0.000609810285548055),(0.,1.),
 .UNSPECIFIED.)
GEOMETRIC_REPRESENTATION_ITEM()
RATIONAL_B_SPLINE_SURFACE(((1.,0.99763002205783,1.),(1.,0.999169954497569,
1.),(1.,1.00000047407105,1.),(1.,1.,1.)))
REPRESENTATION_ITEM('')
SURFACE()
);
#3988=(
BOUNDED_SURFACE()
B_SPLINE_SURFACE(3,2,((#259836,#259837,#259838),(#259839,#259840,#259841),
(#259842,#259843,#259844),(#259845,#259846,#259847),(#259848,#259849,#259850),
(#259851,#259852,#259853),(#259854,#259855,#259856),(#259857,#259858,#259859),
(#259860,#259861,#259862),(#259863,#259864,#259865),(#259866,#259867,#259868),
(#259869,#259870,#259871),(#259872,#259873,#259874),(#259875,#259876,#259877),
(#259878,#259879,#259880),(#259881,#259882,#259883),(#259884,#259885,#259886),
(#259887,#259888,#259889),(#259890,#259891,#259892),(#259893,#259894,#259895),
(#259896,#259897,#259898),(#259899,#259900,#259901),(#259902,#259903,#259904),
(#259905,#259906,#259907),(#259908,#259909,#259910),(#259911,#259912,#259913),
(#259914,#259915,#259916),(#259917,#259918,#259919),(#259920,#259921,#259922),
(#259923,#259924,#259925),(#259926,#259927,#259928),(#259929,#259930,#259931),
(#259932,#259933,#259934),(#259935,#259936,#259937),(#259938,#259939,#259940),
(#259941,#259942,#259943)),.UNSPECIFIED.,.F.,.F.,.F.)
B_SPLINE_SURFACE_WITH_KNOTS((4,2,2,2,2,2,2,2,2,2,2,2,2,2,2,2,2,4),(3,3),
(-0.000333469135128296,0.000833672837820777,0.00166734567564155,0.00250101851346233,
0.00270943672291753,0.00291785493237272,0.00302206403710032,0.00307416858946412,
0.00310022086564602,0.00312627314182791,0.00313929927991886,0.00315232541800981,
0.00316535155610076,0.00317186462514624,0.00317837769419171,0.00320442997037361,
0.00323048224655551,0.00364829276517634),(0.,1.00460570884614),
 .UNSPECIFIED.)
GEOMETRIC_REPRESENTATION_ITEM()
RATIONAL_B_SPLINE_SURFACE(((1.,0.997054706395359,1.00002713032962),(1.,
0.99605271523388,1.00003636008873),(1.,0.994673259186161,1.00004906683457),
(1.,0.992006802794343,1.00007362867816),(1.,0.990790384906993,1.00008483361141),
(1.,0.988393785580759,1.00010690968884),(1.,0.987091346369295,1.00011890700044),
(1.,0.986150203297001,1.00012757626238),(1.,0.986003642672709,1.00012892629351),
(1.,0.98594923782718,1.00012942743927),(1.,0.986000799357347,1.00012895248448),
(1.,0.986777873089688,1.00012179453375),(1.,0.987137483619352,1.00011848201096),
(1.,0.988298093339298,1.00010779115005),(1.,0.988782642230707,1.00010332776782),
(1.,0.989957253593815,1.00009250793192),(1.,0.990423861711881,1.00008820980965),
(1.,0.991688273857576,1.00007656278124),(1.,0.99247603863951,1.00006930635079),
(1.,0.994284431414231,1.00005264848959),(1.,0.995010326911407,1.00004596196297),
(1.,0.996626426244886,1.00003107539697),(1.,0.997501337999239,1.00002301621936),
(1.,0.998874113903667,1.00001037100711),(1.,0.999376314879074,1.00000574502416),
(1.,0.999608475942123,1.00000360649163),(1.,0.999592989064556,1.00000374914773),
(1.,0.999491456297205,1.00000468440846),(1.,0.99940936032604,1.00000544062874),
(1.,0.998997449457976,1.0000092349118),(1.,0.998651286170311,1.00001242356643),
(1.,0.998071024137407,1.00001776860239),(1.,0.997813344969381,1.00002014219284),
(1.,0.993788013597043,1.00005722120146),(1.,0.995307700675226,1.00004322272902),
(0.999999999999997,0.985483842090745,1.00013371439379)))
REPRESENTATION_ITEM('')
SURFACE()
);
#3989=(
BOUNDED_SURFACE()
B_SPLINE_SURFACE(3,2,((#259945,#259946,#259947),(#259948,#259949,#259950),
(#259951,#259952,#259953),(#259954,#259955,#259956)),.UNSPECIFIED.,.F.,
 .F.,.F.)
B_SPLINE_SURFACE_WITH_KNOTS((4,4),(3,3),(-2.85745148645305E-5,0.000314319663509816),
(0.,1.00095479655756),.UNSPECIFIED.)
GEOMETRIC_REPRESENTATION_ITEM()
RATIONAL_B_SPLINE_SURFACE(((1.,0.997737992798767,1.00000431951338),(1.,
0.997316919425135,1.00000512359219),(1.,0.99665184107804,1.00000639362123),
(1.,0.995946994780193,1.00000773959086)))
REPRESENTATION_ITEM('')
SURFACE()
);
#3990=(
BOUNDED_SURFACE()
B_SPLINE_SURFACE(3,2,((#259958,#259959,#259960),(#259961,#259962,#259963),
(#259964,#259965,#259966),(#259967,#259968,#259969)),.UNSPECIFIED.,.F.,
 .F.,.F.)
B_SPLINE_SURFACE_WITH_KNOTS((4,4),(3,3),(-3.03576608295941E-18,0.000609810285535259),
(0.,1.),.UNSPECIFIED.)
GEOMETRIC_REPRESENTATION_ITEM()
RATIONAL_B_SPLINE_SURFACE(((1.,0.997630022057913,1.),(1.,0.999169954497594,
1.),(1.,1.00000047407104,1.),(1.,1.,1.)))
REPRESENTATION_ITEM('')
SURFACE()
);
#3991=(
BOUNDED_SURFACE()
B_SPLINE_SURFACE(3,2,((#259970,#259971,#259972),(#259973,#259974,#259975),
(#259976,#259977,#259978),(#259979,#259980,#259981),(#259982,#259983,#259984),
(#259985,#259986,#259987),(#259988,#259989,#259990),(#259991,#259992,#259993),
(#259994,#259995,#259996),(#259997,#259998,#259999),(#260000,#260001,#260002),
(#260003,#260004,#260005),(#260006,#260007,#260008),(#260009,#260010,#260011),
(#260012,#260013,#260014),(#260015,#260016,#260017),(#260018,#260019,#260020),
(#260021,#260022,#260023),(#260024,#260025,#260026),(#260027,#260028,#260029),
(#260030,#260031,#260032),(#260033,#260034,#260035),(#260036,#260037,#260038),
(#260039,#260040,#260041),(#260042,#260043,#260044),(#260045,#260046,#260047),
(#260048,#260049,#260050),(#260051,#260052,#260053),(#260054,#260055,#260056),
(#260057,#260058,#260059),(#260060,#260061,#260062),(#260063,#260064,#260065),
(#260066,#260067,#260068),(#260069,#260070,#260071),(#260072,#260073,#260074),
(#260075,#260076,#260077),(#260078,#260079,#260080),(#260081,#260082,#260083)),
 .UNSPECIFIED.,.F.,.F.,.F.)
B_SPLINE_SURFACE_WITH_KNOTS((4,2,2,2,2,2,2,2,2,2,2,2,2,2,2,2,2,2,4),(3,
3),(-0.000333361155037782,0.000833402887594952,0.0016668057751899,0.00250020866278486,
0.00270855938468359,0.00291691010658233,0.0030210854675317,0.00307317314800638,
0.00309921698824373,0.00312526082848107,0.00313828274859974,0.00315130466871841,
0.00316432658883708,0.00317083754889642,0.00317734850895575,0.00319037042907442,
0.0032033923491931,0.00322943618943044,0.00364710253335728),(-0.00578770259235711,
1.),.UNSPECIFIED.)
GEOMETRIC_REPRESENTATION_ITEM()
RATIONAL_B_SPLINE_SURFACE(((1.00003412924228,0.997051572559778,1.),(1.00004574779706,
0.996047844863059,1.),(1.00006173418376,0.994666779885507,1.),(1.00009261872355,
0.991998662502961,1.),(1.00010672130462,0.990780339615383,1.),(1.00013449167914,
0.9883812551701,1.),(1.00014956154484,0.987079368501341,1.),(1.00016049009589,
0.986135250271367,1.),(1.00016219281536,0.985988152226901,1.),(1.00016284042277,
0.985932205381424,1.),(1.0001622503025,0.985983185909607,1.),(1.0001533122673,
0.986755343345934,1.),(1.00014917060097,0.987113142167373,1.),(1.00013582833498,
0.988265781386087,1.),(1.00013025774237,0.98874702524063,1.),(1.00011679689681,
0.989909908556455,1.),(1.00011145395186,0.990371485915094,1.),(1.0000970158952,
0.991618790560121,1.),(1.00008804413747,0.99239386128949,1.),(1.0000674722456,
0.99417106835355,1.),(1.0000592294594,0.994883163184569,1.),(1.00004065487868,
0.996487822410277,1.),(1.0000304112453,0.997372770558565,1.),(1.00001405173748,
0.998786069493821,1.),(1.00000795752204,0.999312549158501,1.),(1.00000465267014,
0.999598055526461,1.),(1.00000463105855,0.999599922553604,1.),(1.00000563530084,
0.99951316599758,1.),(1.00000656546673,0.999432808905664,1.),(1.00000942801062,
0.999185513555113,1.),(1.00001147197509,0.999008935332597,1.),(1.00001530309848,
0.998677964335571,1.),(1.00001710470033,0.998522323835872,1.),(1.00002219973076,
0.998082163829078,1.),(1.00002520463239,0.997822570182858,1.),(1.00007209350726,
0.993771837260874,1.),(1.00005489075981,0.99525798372191,1.),(1.00016523340031,
0.985725475896788,1.)))
REPRESENTATION_ITEM('')
SURFACE()
);
#3992=(
BOUNDED_SURFACE()
B_SPLINE_SURFACE(3,2,((#260085,#260086,#260087),(#260088,#260089,#260090),
(#260091,#260092,#260093),(#260094,#260095,#260096)),.UNSPECIFIED.,.F.,
 .F.,.F.)
B_SPLINE_SURFACE_WITH_KNOTS((4,4),(3,3),(-2.85745148634742E-5,0.000314319663498371),
(0.,1.00095479620998),.UNSPECIFIED.)
GEOMETRIC_REPRESENTATION_ITEM()
RATIONAL_B_SPLINE_SURFACE(((1.,0.995946994781608,1.00000773958804),(1.,
0.996651841079179,1.0000063936189),(1.,0.997316919426007,1.00000512359033),
(1.,0.997737992799513,1.0000043195118)))
REPRESENTATION_ITEM('')
SURFACE()
);
#3993=(
BOUNDED_SURFACE()
B_SPLINE_SURFACE(3,2,((#260098,#260099,#260100),(#260101,#260102,#260103),
(#260104,#260105,#260106),(#260107,#260108,#260109)),.UNSPECIFIED.,.F.,
 .F.,.F.)
B_SPLINE_SURFACE_WITH_KNOTS((4,4),(3,3),(2.16840434497101E-19,0.000609810285548116),
(0.,1.),.UNSPECIFIED.)
GEOMETRIC_REPRESENTATION_ITEM()
RATIONAL_B_SPLINE_SURFACE(((1.,0.99763002205783,1.),(1.,0.999169954497568,
1.),(1.,1.00000047407105,1.),(1.,1.,1.)))
REPRESENTATION_ITEM('')
SURFACE()
);
#3994=(
BOUNDED_SURFACE()
B_SPLINE_SURFACE(3,2,((#260110,#260111,#260112),(#260113,#260114,#260115),
(#260116,#260117,#260118),(#260119,#260120,#260121),(#260122,#260123,#260124),
(#260125,#260126,#260127),(#260128,#260129,#260130),(#260131,#260132,#260133),
(#260134,#260135,#260136),(#260137,#260138,#260139),(#260140,#260141,#260142),
(#260143,#260144,#260145),(#260146,#260147,#260148),(#260149,#260150,#260151),
(#260152,#260153,#260154),(#260155,#260156,#260157),(#260158,#260159,#260160),
(#260161,#260162,#260163),(#260164,#260165,#260166),(#260167,#260168,#260169),
(#260170,#260171,#260172),(#260173,#260174,#260175),(#260176,#260177,#260178),
(#260179,#260180,#260181),(#260182,#260183,#260184),(#260185,#260186,#260187),
(#260188,#260189,#260190),(#260191,#260192,#260193),(#260194,#260195,#260196),
(#260197,#260198,#260199),(#260200,#260201,#260202),(#260203,#260204,#260205),
(#260206,#260207,#260208),(#260209,#260210,#260211),(#260212,#260213,#260214),
(#260215,#260216,#260217)),.UNSPECIFIED.,.F.,.F.,.F.)
B_SPLINE_SURFACE_WITH_KNOTS((4,2,2,2,2,2,2,2,2,2,2,2,2,2,2,2,2,4),(3,3),
(0.,0.000833672837821486,0.00166734567564297,0.00250101851346446,0.00270943672291983,
0.0029178549323752,0.00302206403710289,0.00307416858946673,0.00310022086564865,
0.00312627314183057,0.00313929927992153,0.00315232541801249,0.00316535155610345,
0.00317186462514893,0.00317837769419441,0.00320442997037634,0.00323048224655826,
0.00364829276517993),(0.,1.00358549869618),.UNSPECIFIED.)
GEOMETRIC_REPRESENTATION_ITEM()
RATIONAL_B_SPLINE_SURFACE(((1.,0.99611206821392,1.0000278803487),(1.,0.995254912868937,
1.00003402700744),(1.,0.994234710580471,1.00004134287539),(1.,0.992014920149054,
1.00005726098679),(1.,0.990799737574257,1.00006597505786),(1.,0.988405572073208,
1.00008314361243),(1.,0.987104455530704,1.00009247391576),(1.,0.986164268221475,
1.00009921599651),(1.,0.986017856433839,1.00010026591505),(1.,0.985963506838659,
1.00010065565586),(1.,0.986015016006277,1.00010028628375),(1.,0.986791300594523,
1.00009471954899),(1.,0.987150545928039,1.00009214340164),(1.,0.9883099770105,
1.00008382912437),(1.,0.988794033826467,1.00008035795421),(1.,0.989967452333396,
1.00007194337316),(1.,0.990433586595655,1.00006860072558),(1.,0.991696714688982,
1.00005954283731),(1.,0.992483679469992,1.00005389951492),(1.,0.994290235762475,
1.00004094470446),(1.,0.995015394088985,1.00003574459599),(1.,0.99662985222034,
1.00002416732094),(1.,0.997503875472981,1.00001789970247),(1.,0.998875257278488,
1.00000806552712),(1.,0.999376948252015,1.00000446790246),(1.,0.999608873547708,
1.00000280476677),(1.,0.999593402397524,1.00000291571035),(1.,0.999491972739996,
1.00000364306216),(1.,0.999409960139993,1.0000042311743),(1.,0.998998467580922,
1.00000718198637),(1.,0.998652655833498,1.0000096618015),(1.,0.998072983075812,
1.00001381863334),(1.,0.997815565589447,1.00001566457346),(1.,0.993794322073923,
1.00004450090023),(1.,0.995312465856801,1.00003361429512),(1.,0.985498583743996,
1.00010398961816)))
REPRESENTATION_ITEM('')
SURFACE()
);
#3995=(
BOUNDED_SURFACE()
B_SPLINE_SURFACE(3,2,((#260219,#260220,#260221),(#260222,#260223,#260224),
(#260225,#260226,#260227),(#260228,#260229,#260230)),.UNSPECIFIED.,.F.,
 .F.,.F.)
B_SPLINE_SURFACE_WITH_KNOTS((4,4),(3,3),(-2.85745148645381E-5,0.000314319663509926),
(0.,1.00095479654686),.UNSPECIFIED.)
GEOMETRIC_REPRESENTATION_ITEM()
RATIONAL_B_SPLINE_SURFACE(((1.,0.997737992798791,1.00000431951333),(1.,
0.997316919425162,1.00000512359214),(1.,0.996651841078075,1.00000639362115),
(1.,0.995946994780235,1.00000773959078)))
REPRESENTATION_ITEM('')
SURFACE()
);
#3996=(
BOUNDED_SURFACE()
B_SPLINE_SURFACE(3,2,((#260232,#260233,#260234),(#260235,#260236,#260237),
(#260238,#260239,#260240),(#260241,#260242,#260243)),.UNSPECIFIED.,.F.,
 .F.,.F.)
B_SPLINE_SURFACE_WITH_KNOTS((4,4),(3,3),(-1.30104260698261E-17,0.00060981028553535),
(0.,1.),.UNSPECIFIED.)
GEOMETRIC_REPRESENTATION_ITEM()
RATIONAL_B_SPLINE_SURFACE(((1.,0.997630022057914,1.),(1.,0.999169954497593,
1.),(1.,1.00000047407104,1.),(1.,1.,1.)))
REPRESENTATION_ITEM('')
SURFACE()
);
#3997=(
BOUNDED_SURFACE()
B_SPLINE_SURFACE(3,2,((#260244,#260245,#260246),(#260247,#260248,#260249),
(#260250,#260251,#260252),(#260253,#260254,#260255),(#260256,#260257,#260258),
(#260259,#260260,#260261),(#260262,#260263,#260264),(#260265,#260266,#260267),
(#260268,#260269,#260270),(#260271,#260272,#260273),(#260274,#260275,#260276),
(#260277,#260278,#260279),(#260280,#260281,#260282),(#260283,#260284,#260285),
(#260286,#260287,#260288),(#260289,#260290,#260291),(#260292,#260293,#260294),
(#260295,#260296,#260297),(#260298,#260299,#260300),(#260301,#260302,#260303),
(#260304,#260305,#260306),(#260307,#260308,#260309),(#260310,#260311,#260312),
(#260313,#260314,#260315),(#260316,#260317,#260318),(#260319,#260320,#260321),
(#260322,#260323,#260324),(#260325,#260326,#260327),(#260328,#260329,#260330),
(#260331,#260332,#260333),(#260334,#260335,#260336),(#260337,#260338,#260339),
(#260340,#260341,#260342),(#260343,#260344,#260345),(#260346,#260347,#260348),
(#260349,#260350,#260351),(#260352,#260353,#260354),(#260355,#260356,#260357)),
 .UNSPECIFIED.,.F.,.F.,.F.)
B_SPLINE_SURFACE_WITH_KNOTS((4,2,2,2,2,2,2,2,2,2,2,2,2,2,2,2,2,2,4),(3,
3),(0.,0.000833402889145506,0.00166680577829101,0.00250020866743652,0.0027085593897229,
0.00291691011200927,0.00302108547315246,0.00307317315372405,0.00309921699400985,
0.00312526083429565,0.00313828275443855,0.00315130467458145,0.00316432659472434,
0.00317083755479579,0.00317734851486724,0.00319037043501014,0.00320339235515304,
0.00322943619543884,0.00364710254014991),(-0.000788950096851769,1.),
 .UNSPECIFIED.)
GEOMETRIC_REPRESENTATION_ITEM()
RATIONAL_B_SPLINE_SURFACE(((1.00000611767343,0.996122902159017,1.),(1.00000746664395,
0.99526798717725,1.),(1.00000907164837,0.994250809774906,1.),(1.00001256256436,
0.992038429042989,1.),(1.00001447540202,0.990826161202841,1.),(1.00001824210387,
0.988439000173286,1.),(1.00002028614152,0.987143583861509,1.),(1.00002176846193,
0.986204157895867,1.),(1.00002199941439,0.986057790929556,1.),(1.00002208725417,
0.986002122151637,1.),(1.00002200721177,0.986052849314101,1.),(1.0000207948797,
0.986821169180919,1.),(1.00002023311476,0.987177189764058,1.),(1.00001842340415,
0.988324100457808,1.),(1.00001766782331,0.988802952568642,1.),(1.00001584202883,
0.98996005647675,1.),(1.00001511732551,0.990419339847295,1.),(1.00001315898457,
0.991660445556412,1.),(1.00001194207836,0.992431664304351,1.),(1.00000915175965,
0.99420003895694,1.),(1.00000803372924,0.994908594810006,1.),(1.0000055143209,
0.996505279029039,1.),(1.00000412490098,0.997385828969795,1.),(1.00000190594012,
0.998792103501718,1.),(1.00000107933685,0.999315966336424,1.),(1.00000063107598,
0.999600053297392,1.),(1.00000062814488,0.999601910890056,1.),(1.00000076435795,
0.999515585363006,1.),(1.00000089052328,0.999435627624268,1.),(1.00000127879138,
0.999189561299934,1.),(1.00000155602942,0.999013860679829,1.),(1.00000207567308,
0.998684534617987,1.),(1.00000232003768,0.998529667660177,1.),(1.00000301111441,
0.998091695265869,1.),(1.00000341869149,0.99783339180862,1.),(1.00000977857705,
0.993802791147178,1.),(1.00000744524123,0.995281551233468,1.),(1.00002241183025,
0.985796420873754,0.999999999999997)))
REPRESENTATION_ITEM('')
SURFACE()
);
#3998=(
BOUNDED_SURFACE()
B_SPLINE_SURFACE(3,2,((#260359,#260360,#260361),(#260362,#260363,#260364),
(#260365,#260366,#260367),(#260368,#260369,#260370)),.UNSPECIFIED.,.F.,
 .F.,.F.)
B_SPLINE_SURFACE_WITH_KNOTS((4,4),(3,3),(-2.8574514863482E-5,0.000314319663498302),
(0.,1.00095479615814),.UNSPECIFIED.)
GEOMETRIC_REPRESENTATION_ITEM()
RATIONAL_B_SPLINE_SURFACE(((1.,0.995946994781818,1.00000773958762),(1.,
0.996651841079349,1.00000639361855),(1.,0.997316919426149,1.00000512359005),
(1.,0.997737992799628,1.00000431951157)))
REPRESENTATION_ITEM('')
SURFACE()
);
#3999=(
BOUNDED_SURFACE()
B_SPLINE_SURFACE(3,2,((#260372,#260373,#260374),(#260375,#260376,#260377),
(#260378,#260379,#260380),(#260381,#260382,#260383)),.UNSPECIFIED.,.F.,
 .F.,.F.)
B_SPLINE_SURFACE_WITH_KNOTS((4,4),(3,3),(2.16840434497101E-19,0.000609810285548094),
(0.,1.),.UNSPECIFIED.)
GEOMETRIC_REPRESENTATION_ITEM()
RATIONAL_B_SPLINE_SURFACE(((1.,0.997630022057829,1.),(1.,0.999169954497567,
1.),(1.,1.00000047407105,1.),(1.,1.,1.)))
REPRESENTATION_ITEM('')
SURFACE()
);
#4000=(
BOUNDED_SURFACE()
B_SPLINE_SURFACE(3,2,((#260384,#260385,#260386),(#260387,#260388,#260389),
(#260390,#260391,#260392),(#260393,#260394,#260395),(#260396,#260397,#260398),
(#260399,#260400,#260401),(#260402,#260403,#260404),(#260405,#260406,#260407),
(#260408,#260409,#260410),(#260411,#260412,#260413),(#260414,#260415,#260416),
(#260417,#260418,#260419),(#260420,#260421,#260422),(#260423,#260424,#260425),
(#260426,#260427,#260428),(#260429,#260430,#260431),(#260432,#260433,#260434),
(#260435,#260436,#260437),(#260438,#260439,#260440),(#260441,#260442,#260443),
(#260444,#260445,#260446),(#260447,#260448,#260449),(#260450,#260451,#260452),
(#260453,#260454,#260455),(#260456,#260457,#260458),(#260459,#260460,#260461),
(#260462,#260463,#260464),(#260465,#260466,#260467),(#260468,#260469,#260470),
(#260471,#260472,#260473),(#260474,#260475,#260476),(#260477,#260478,#260479),
(#260480,#260481,#260482),(#260483,#260484,#260485),(#260486,#260487,#260488),
(#260489,#260490,#260491)),.UNSPECIFIED.,.F.,.F.,.F.)
B_SPLINE_SURFACE_WITH_KNOTS((4,2,2,2,2,2,2,2,2,2,2,2,2,2,2,2,2,4),(3,3),
(-0.0003334691351286,0.000833672837821643,0.00166734567564329,0.00250101851346493,
0.00270943672292034,0.00291785493237575,0.00302206403710345,0.00307416858946731,
0.00310022086564923,0.00312627314183116,0.00313929927992212,0.00315232541801309,
0.00316535155610405,0.00317186462514953,0.00317837769419501,0.00320442997037694,
0.00323048224655887,0.00364829276517932),(0.,1.00460570885116),
 .UNSPECIFIED.)
GEOMETRIC_REPRESENTATION_ITEM()
RATIONAL_B_SPLINE_SURFACE(((1.,0.99705470639553,1.00002713032965),(1.,0.996052715233661,
1.00003636008877),(1.,0.99467325918624,1.00004906683463),(1.,0.99200680279422,
1.00007362867824),(1.,0.990790384906983,1.0000848336115),(1.,0.988393785580642,
1.00010690968896),(1.,0.987091346368492,1.00011890700057),(1.,0.986150203297094,
1.00012757626252),(1.,0.986003642672512,1.00012892629365),(1.,0.985949237827209,
1.00012942743941),(1.,0.986000799357252,1.00012895248462),(1.,0.986777873089627,
1.00012179453388),(1.,0.987137483619315,1.00011848201109),(1.,0.988298093339291,
1.00010779115017),(1.,0.98878264223078,1.00010332776793),(1.,0.989957253593888,
1.00009250793203),(1.,0.990423861712164,1.00008820980974),(1.,0.991688273857629,
1.00007656278132),(1.,0.992476038639695,1.00006930635087),(1.,0.994284431414586,
1.00005264848965),(1.,0.995010326911815,1.00004596196301),(1.,0.996626426245307,
1.000031075397),(1.,0.99750133799964,1.00002301621938),(1.,0.998874113904101,
1.00001037100711),(1.,0.999376314879296,1.00000574502416),(1.,0.999608475942149,
1.00000360649164),(1.,0.999592989064516,1.00000374914774),(1.,0.999491456297114,
1.00000468440847),(1.,0.99940936032594,1.00000544062875),(1.,0.998997449457861,
1.00000923491181),(1.,0.99865128617018,1.00001242356645),(1.,0.998071024137341,
1.00001776860241),(1.,0.997813344969334,1.00002014219286),(1.,0.993788013596569,
1.00005722120152),(1.,0.995307700678994,1.00004322272903),(1.,0.985483842068487,
1.00013371439414)))
REPRESENTATION_ITEM('')
SURFACE()
);
#4001=(
BOUNDED_SURFACE()
B_SPLINE_SURFACE(3,2,((#260493,#260494,#260495),(#260496,#260497,#260498),
(#260499,#260500,#260501),(#260502,#260503,#260504)),.UNSPECIFIED.,.F.,
 .F.,.F.)
B_SPLINE_SURFACE_WITH_KNOTS((4,4),(3,3),(-2.85745148645395E-5,0.000314319663509989),
(0.,1.00095479660429),.UNSPECIFIED.)
GEOMETRIC_REPRESENTATION_ITEM()
RATIONAL_B_SPLINE_SURFACE(((1.,0.997737992798662,1.00000431951359),(1.,
0.997316919425008,1.00000512359244),(1.,0.996651841077884,1.00000639362154),
(1.,0.995946994780003,1.00000773959124)))
REPRESENTATION_ITEM('')
SURFACE()
);
#4002=(
BOUNDED_SURFACE()
B_SPLINE_SURFACE(3,2,((#260506,#260507,#260508),(#260509,#260510,#260511),
(#260512,#260513,#260514),(#260515,#260516,#260517)),.UNSPECIFIED.,.F.,
 .F.,.F.)
B_SPLINE_SURFACE_WITH_KNOTS((4,4),(3,3),(-4.77048955893622E-18,0.000609810285535309),
(0.,1.),.UNSPECIFIED.)
GEOMETRIC_REPRESENTATION_ITEM()
RATIONAL_B_SPLINE_SURFACE(((1.,0.997630022057914,1.),(1.,0.999169954497594,
1.),(1.,1.00000047407104,1.),(1.,1.,1.)))
REPRESENTATION_ITEM('')
SURFACE()
);
#4003=(
BOUNDED_SURFACE()
B_SPLINE_SURFACE(3,2,((#260518,#260519,#260520),(#260521,#260522,#260523),
(#260524,#260525,#260526),(#260527,#260528,#260529)),.UNSPECIFIED.,.F.,
 .F.,.F.)
B_SPLINE_SURFACE_WITH_KNOTS((4,4),(3,3),(0.,0.000609810285548325),(0.,1.),
 .UNSPECIFIED.)
GEOMETRIC_REPRESENTATION_ITEM()
RATIONAL_B_SPLINE_SURFACE(((1.,0.997630022057829,1.),(1.,0.999169954497567,
1.),(1.,1.00000047407105,1.),(1.,1.,1.)))
REPRESENTATION_ITEM('')
SURFACE()
);
#4004=(
BOUNDED_SURFACE()
B_SPLINE_SURFACE(3,2,((#260531,#260532,#260533),(#260534,#260535,#260536),
(#260537,#260538,#260539),(#260540,#260541,#260542)),.UNSPECIFIED.,.F.,
 .F.,.F.)
B_SPLINE_SURFACE_WITH_KNOTS((4,4),(3,3),(-2.85745148634637E-5,0.000314319663498177),
(0.,1.00095479624155),.UNSPECIFIED.)
GEOMETRIC_REPRESENTATION_ITEM()
RATIONAL_B_SPLINE_SURFACE(((1.,0.995946994781479,1.0000077395883),(1.,0.996651841079075,
1.00000639361911),(1.,0.997316919425921,1.0000051235905),(1.,0.997737992799442,
1.00000431951195)))
REPRESENTATION_ITEM('')
SURFACE()
);
#4005=(
BOUNDED_SURFACE()
B_SPLINE_SURFACE(3,2,((#260544,#260545,#260546),(#260547,#260548,#260549),
(#260550,#260551,#260552),(#260553,#260554,#260555),(#260556,#260557,#260558),
(#260559,#260560,#260561),(#260562,#260563,#260564),(#260565,#260566,#260567),
(#260568,#260569,#260570),(#260571,#260572,#260573),(#260574,#260575,#260576),
(#260577,#260578,#260579),(#260580,#260581,#260582),(#260583,#260584,#260585),
(#260586,#260587,#260588),(#260589,#260590,#260591),(#260592,#260593,#260594),
(#260595,#260596,#260597),(#260598,#260599,#260600),(#260601,#260602,#260603),
(#260604,#260605,#260606),(#260607,#260608,#260609),(#260610,#260611,#260612),
(#260613,#260614,#260615),(#260616,#260617,#260618),(#260619,#260620,#260621),
(#260622,#260623,#260624),(#260625,#260626,#260627),(#260628,#260629,#260630),
(#260631,#260632,#260633),(#260634,#260635,#260636),(#260637,#260638,#260639),
(#260640,#260641,#260642),(#260643,#260644,#260645),(#260646,#260647,#260648),
(#260649,#260650,#260651),(#260652,#260653,#260654),(#260655,#260656,#260657)),
 .UNSPECIFIED.,.F.,.F.,.F.)
B_SPLINE_SURFACE_WITH_KNOTS((4,2,2,2,2,2,2,2,2,2,2,2,2,2,2,2,2,2,4),(3,
3),(-0.000333361155718326,0.000833402889296124,0.00166680577859225,0.00250020866788837,
0.0027085593902124,0.00291691011253643,0.00302108547369845,0.00307317315427946,
0.00309921699456996,0.00312526083486046,0.00313828275500572,0.00315130467515097,
0.00316432659529622,0.00317083755536884,0.00317734851544147,0.00319037043558672,
0.00320339235573198,0.00322943619602248,0.00364710254080976),(-0.00578770663227079,
1.),.UNSPECIFIED.)
GEOMETRIC_REPRESENTATION_ITEM()
RATIONAL_B_SPLINE_SURFACE(((1.00003412926621,0.997051572550087,1.),(1.00004574782918,
0.996047844846918,1.),(1.00006173422714,0.994666779861184,1.),(1.00009261878868,
0.991998662461224,1.),(1.00010672137968,0.990780339566208,1.),(1.00013449177376,
0.988381255106199,1.),(1.00014956165008,0.98707936842808,1.),(1.0001604902087,
0.986135250203682,1.),(1.00016219292933,0.985988152161554,1.),(1.00016284053703,
0.98593220532956,1.),(1.00016225041626,0.98598318586536,1.),(1.00015331237424,
0.986755343352947,1.),(1.00014917070478,0.987113142194872,1.),(1.00013582842843,
0.988265781504093,1.),(1.0001302578315,0.988747025396118,1.),(1.0001167969751,
0.989909908835822,1.),(1.00011145402582,0.990371486246688,1.),(1.00009701595708,
0.991618791065173,1.),(1.00008804419163,0.992393861919777,1.),(1.00006747228168,
0.994171069305731,1.),(1.0000592294881,0.994883164277001,1.),(1.00004065489268,
0.996487823652573,1.),(1.00003041125244,0.997372771775525,1.),(1.00001405173728,
0.998786070358076,1.),(1.00000795752053,0.999312549768481,1.),(1.00000465267198,
0.999598055648167,1.),(1.00000463106235,0.999599922504002,1.),(1.00000563530726,
0.999513165782186,1.),(1.00000656547408,0.999432808667257,1.),(1.00000942802033,
0.99918551328416,1.),(1.0000114719861,0.999008935072858,1.),(1.00001530311202,
0.998677964089285,1.),(1.00001710471499,0.998522323600551,1.),(1.00002219974871,
0.998082163617035,1.),(1.00002520465231,0.997822569982669,1.),(1.00007209355794,
0.993771837229935,1.),(1.0000548908016,0.995257983422156,1.),(1.00016523350623,
0.985725476710866,1.)))
REPRESENTATION_ITEM('')
SURFACE()
);
#4006=(
BOUNDED_SURFACE()
B_SPLINE_SURFACE(3,2,((#260658,#260659,#260660),(#260661,#260662,#260663),
(#260664,#260665,#260666),(#260667,#260668,#260669),(#260670,#260671,#260672),
(#260673,#260674,#260675),(#260676,#260677,#260678),(#260679,#260680,#260681),
(#260682,#260683,#260684),(#260685,#260686,#260687),(#260688,#260689,#260690),
(#260691,#260692,#260693),(#260694,#260695,#260696),(#260697,#260698,#260699),
(#260700,#260701,#260702),(#260703,#260704,#260705),(#260706,#260707,#260708),
(#260709,#260710,#260711),(#260712,#260713,#260714),(#260715,#260716,#260717),
(#260718,#260719,#260720),(#260721,#260722,#260723),(#260724,#260725,#260726),
(#260727,#260728,#260729),(#260730,#260731,#260732),(#260733,#260734,#260735),
(#260736,#260737,#260738),(#260739,#260740,#260741),(#260742,#260743,#260744),
(#260745,#260746,#260747),(#260748,#260749,#260750),(#260751,#260752,#260753),
(#260754,#260755,#260756),(#260757,#260758,#260759),(#260760,#260761,#260762),
(#260763,#260764,#260765)),.UNSPECIFIED.,.F.,.F.,.F.)
B_SPLINE_SURFACE_WITH_KNOTS((4,2,2,2,2,2,2,2,2,2,2,2,2,2,2,2,2,4),(3,3),
(-0.000333469135129058,0.000833672837822158,0.00166734567564438,0.00250101851346661,
0.00270943672292216,0.00291785493237772,0.0030220640371055,0.00307416858946939,
0.00310022086565133,0.00312627314183328,0.00313929927992425,0.00315232541801522,
0.00316535155610619,0.00317186462515168,0.00317837769419717,0.00320442997037911,
0.00323048224656105,0.00364829276518163),(0.,1.0046057089022),
 .UNSPECIFIED.)
GEOMETRIC_REPRESENTATION_ITEM()
RATIONAL_B_SPLINE_SURFACE(((1.,0.997054706395145,1.00002713032995),(1.,
0.996052715233707,1.00003636008918),(1.,0.994673259185837,1.00004906683517),
(1.,0.992006802793903,1.00007362867906),(1.,0.990790384906695,1.00008483361244),
(1.,0.988393785579858,1.00010690969015),(1.,0.987091346368048,1.0001189070019),
(1.,0.986150203296328,1.00012757626394),(1.,0.986003642671745,1.00012892629509),
(1.,0.985949237826535,1.00012942744085),(1.,0.986000799356981,1.00012895248605),
(1.,0.98677787308873,1.00012179453524),(1.,0.987137483618698,1.0001184820124),
(1.,0.988298093338714,1.00010779115137),(1.,0.988782642230273,1.00010332776908),
(1.,0.989957253593439,1.00009250793305),(1.,0.990423861711556,1.00008820981073),
(1.,0.99168827385752,1.00007656278217),(1.,0.992476038639505,1.00006930635164),
(1.,0.994284431414554,1.00005264849023),(1.,0.995010326911985,1.00004596196352),
(1.,0.996626426245523,1.00003107539735),(1.,0.997501337999955,1.00002301621963),
(1.,0.998874113904281,1.00001037100723),(1.,0.999376314879437,1.00000574502422),
(1.,0.99960847594215,1.00000360649168),(1.,0.999592989064471,1.00000374914778),
(1.,0.999491456297019,1.00000468440852),(1.,0.999409360325836,1.00000544062881),
(1.,0.998997449457727,1.00000923491191),(1.,0.998651286170026,1.00001242356659),
(1.,0.998071024137219,1.00001776860261),(1.,0.997813344969144,1.00002014219308),
(1.,0.993788013596835,1.00005722120215),(1.,0.995307700673881,1.00004322272956),
(1.,0.985483842096778,1.00013371439536)))
REPRESENTATION_ITEM('')
SURFACE()
);
#4007=(
BOUNDED_SURFACE()
B_SPLINE_SURFACE(3,2,((#260767,#260768,#260769),(#260770,#260771,#260772),
(#260773,#260774,#260775),(#260776,#260777,#260778)),.UNSPECIFIED.,.F.,
 .F.,.F.)
B_SPLINE_SURFACE_WITH_KNOTS((4,4),(3,3),(-2.85745148645424E-5,0.000314319663509999),
(0.,1.00095479657711),.UNSPECIFIED.)
GEOMETRIC_REPRESENTATION_ITEM()
RATIONAL_B_SPLINE_SURFACE(((1.,0.997737992798722,1.00000431951347),(1.,
0.997316919425082,1.0000051235923),(1.,0.996651841077974,1.00000639362136),
(1.,0.995946994780112,1.00000773959102)))
REPRESENTATION_ITEM('')
SURFACE()
);
#4008=(
BOUNDED_SURFACE()
B_SPLINE_SURFACE(3,2,((#260780,#260781,#260782),(#260783,#260784,#260785),
(#260786,#260787,#260788),(#260789,#260790,#260791)),.UNSPECIFIED.,.F.,
 .F.,.F.)
B_SPLINE_SURFACE_WITH_KNOTS((4,4),(3,3),(-1.23599047663348E-17,0.000609810285535295),
(0.,1.),.UNSPECIFIED.)
GEOMETRIC_REPRESENTATION_ITEM()
RATIONAL_B_SPLINE_SURFACE(((1.,0.997630022057914,1.),(1.,0.999169954497594,
1.),(1.,1.00000047407104,1.),(1.,1.,1.)))
REPRESENTATION_ITEM('')
SURFACE()
);
#4009=(
BOUNDED_SURFACE()
B_SPLINE_SURFACE(3,2,((#260792,#260793,#260794),(#260795,#260796,#260797),
(#260798,#260799,#260800),(#260801,#260802,#260803),(#260804,#260805,#260806),
(#260807,#260808,#260809),(#260810,#260811,#260812),(#260813,#260814,#260815),
(#260816,#260817,#260818),(#260819,#260820,#260821),(#260822,#260823,#260824),
(#260825,#260826,#260827),(#260828,#260829,#260830),(#260831,#260832,#260833)),
 .UNSPECIFIED.,.F.,.F.,.F.)
B_SPLINE_SURFACE_WITH_KNOTS((4,2,2,2,2,2,4),(3,3),(-1.73472347597681E-18,
0.00136118311773746,0.00204177467660619,0.00272236623547492,0.00340295779434365,
0.00408354935321238,0.00544473247094984),(0.,1.),.UNSPECIFIED.)
GEOMETRIC_REPRESENTATION_ITEM()
RATIONAL_B_SPLINE_SURFACE(((1.,0.748955720789002,1.),(1.,0.74826415820711,
1.),(1.,0.746711680960384,1.),(1.,0.74314634401593,1.),(1.,0.741776455602707,
1.),(1.,0.738679679513325,1.),(1.,0.736933927001107,1.),(1.,0.733153776741552,
1.),(1.,0.731132725915841,1.),(1.,0.726827414419606,1.),(1.,0.724518460380596,
1.),(1.,0.717397817977927,1.),(1.,0.71235845960716,1.),(1.,0.707106781186548,
1.)))
REPRESENTATION_ITEM('')
SURFACE()
);
#4010=(
BOUNDED_SURFACE()
B_SPLINE_SURFACE(3,2,((#260850,#260851,#260852),(#260853,#260854,#260855),
(#260856,#260857,#260858),(#260859,#260860,#260861),(#260862,#260863,#260864),
(#260865,#260866,#260867),(#260868,#260869,#260870),(#260871,#260872,#260873),
(#260874,#260875,#260876),(#260877,#260878,#260879),(#260880,#260881,#260882),
(#260883,#260884,#260885),(#260886,#260887,#260888),(#260889,#260890,#260891)),
 .UNSPECIFIED.,.F.,.F.,.F.)
B_SPLINE_SURFACE_WITH_KNOTS((4,2,2,2,2,2,4),(3,3),(0.,0.00136134654673614,
0.00204201982010421,0.00272269309347228,0.00340336636684036,0.00408403964020843,
0.00544538618694457),(0.,1.),.UNSPECIFIED.)
GEOMETRIC_REPRESENTATION_ITEM()
RATIONAL_B_SPLINE_SURFACE(((1.,0.707106781186547,1.),(1.,0.712303169346064,
1.),(1.,0.717355648681421,1.),(1.,0.724523494465793,1.),(1.,0.726790378288212,
1.),(1.,0.731092716345856,1.),(1.,0.733143854998034,1.),(1.,0.736930899570443,
1.),(1.,0.738649526515843,1.),(1.,0.741751075820653,1.),(1.,0.743145323860387,
1.),(1.,0.746698948407202,1.),(1.,0.748249049712917,1.),(1.,0.748955720789002,
1.)))
REPRESENTATION_ITEM('')
SURFACE()
);
#4011=(
BOUNDED_SURFACE()
B_SPLINE_SURFACE(3,2,((#260929,#260930,#260931),(#260932,#260933,#260934),
(#260935,#260936,#260937),(#260938,#260939,#260940),(#260941,#260942,#260943),
(#260944,#260945,#260946),(#260947,#260948,#260949),(#260950,#260951,#260952),
(#260953,#260954,#260955),(#260956,#260957,#260958),(#260959,#260960,#260961),
(#260962,#260963,#260964),(#260965,#260966,#260967),(#260968,#260969,#260970),
(#260971,#260972,#260973),(#260974,#260975,#260976),(#260977,#260978,#260979),
(#260980,#260981,#260982),(#260983,#260984,#260985),(#260986,#260987,#260988),
(#260989,#260990,#260991),(#260992,#260993,#260994)),.UNSPECIFIED.,.F.,
 .F.,.F.)
B_SPLINE_SURFACE_WITH_KNOTS((4,2,2,2,2,2,2,2,2,2,4),(3,3),(-5.08913310798276E-12,
0.000351116935758021,0.000526675406181597,0.000702233876605174,0.00105335081745233,
0.00140446775829948,0.00175558469914664,0.00193114316957021,0.00210670163999379,
0.00245781858084094,0.0028089355216881),(0.,1.00212154420491),
 .UNSPECIFIED.)
GEOMETRIC_REPRESENTATION_ITEM()
RATIONAL_B_SPLINE_SURFACE(((1.,0.981880755432236,1.00007688155662),(1.,
0.981882092332791,1.00007687588403),(1.,0.981880407724475,1.00007688303197),
(1.,0.981878412726316,1.00007689149693),(1.,0.98187708093562,1.00007689714783),
(1.,0.981874393254514,1.0000769085519),(1.,0.981872947013521,1.00007691468843),
(1.,0.981868716388952,1.00007693263935),(1.,0.981866966616579,1.00007694006378),
(1.,0.98186071974881,1.0000769665698),(1.,0.981861064282868,1.00007696510791),
(1.,0.981858769625711,1.00007697484434),(1.,0.981858540956784,1.0000769758146),
(1.,0.981862047984854,1.00007696093397),(1.,0.981862448285702,1.00007695923546),
(1.,0.981864314970464,1.00007695131495),(1.,0.981865383122516,1.00007694678269),
(1.,0.981869817883337,1.00007692796561),(1.,0.98187226500369,1.00007691758226),
(1.,0.98187820748076,1.0000768923678),(1.,0.981879815049627,1.00007688554675),
(1.,0.98188078670202,1.00007688142394)))
REPRESENTATION_ITEM('')
SURFACE()
);
#4012=(
BOUNDED_SURFACE()
B_SPLINE_SURFACE(3,2,((#261416,#261417,#261418),(#261419,#261420,#261421),
(#261422,#261423,#261424),(#261425,#261426,#261427),(#261428,#261429,#261430),
(#261431,#261432,#261433),(#261434,#261435,#261436),(#261437,#261438,#261439),
(#261440,#261441,#261442),(#261443,#261444,#261445),(#261446,#261447,#261448),
(#261449,#261450,#261451),(#261452,#261453,#261454),(#261455,#261456,#261457),
(#261458,#261459,#261460),(#261461,#261462,#261463),(#261464,#261465,#261466),
(#261467,#261468,#261469),(#261470,#261471,#261472),(#261473,#261474,#261475)),
 .UNSPECIFIED.,.F.,.F.,.F.)
B_SPLINE_SURFACE_WITH_KNOTS((4,2,2,2,2,2,2,2,2,4),(3,3),(0.0026254766208179,
0.00351116940646127,0.0038622863488768,0.00403784482008456,0.00421340329129233,
0.00456452023370786,0.00491563717612339,0.00509119564733115,0.00526675411853892,
0.00589876461495421),(-0.00125569467631438,1.00180257992218),
 .UNSPECIFIED.)
GEOMETRIC_REPRESENTATION_ITEM()
RATIONAL_B_SPLINE_SURFACE(((1.00004547719783,0.981858935225732,1.00006531926962),
(1.00004544657458,0.981871150982356,1.00006527528519),(1.00004547473781,
0.981859916538268,1.00006531573627),(1.00004549367077,0.981852364094264,
1.00006534292983),(1.00004550322764,0.981848551814997,1.00006535665644),
(1.00004551019068,0.981845774225094,1.00006536665751),(1.00004551240719,
0.981844890048581,1.00006536984111),(1.00004551592272,0.981843487685747,
1.0000653748905),(1.00004551706357,0.981843032597144,1.0000653765291),(1.00004551844175,
0.981842482833192,1.0000653785086),(1.00004551600531,0.981843454742648,
1.00006537500911),(1.00004551339811,0.981844494765837,1.00006537126438),
(1.00004550803579,0.981846633818991,1.00006536356243),(1.00004549615002,
0.981851375109875,1.0000653464908),(1.00004549312932,0.981852580080655,
1.00006534215214),(1.00004548600682,0.981855421277189,1.00006533192205),
(1.0000454836188,0.981856373870441,1.00006532849211),(1.00004546289328,
0.981864641377868,1.00006529872387),(1.00004547077922,0.981861495638696,
1.00006531005052),(1.00004544888931,0.981870227625078,1.00006527860986)))
REPRESENTATION_ITEM('')
SURFACE()
);
#4013=(
BOUNDED_SURFACE()
B_SPLINE_SURFACE(1,2,((#262489,#262490,#262491,#262492,#262493,#262494,
#262495,#262496,#262497,#262498,#262499,#262500,#262501,#262502,#262503,
#262504,#262505,#262506,#262507,#262508,#262509,#262510,#262511,#262512,
#262513,#262514,#262515,#262516,#262517,#262518,#262519,#262520,#262521,
#262522,#262523,#262524,#262525,#262526,#262527,#262528,#262529,#262530,
#262531,#262532,#262533,#262534,#262535,#262536,#262537,#262538,#262539,
#262540,#262541,#262542,#262543,#262544,#262545,#262546,#262547,#262548,
#262549,#262550,#262551,#262552,#262553,#262554,#262555,#262556,#262557,
#262558,#262559,#262560,#262561,#262562,#262563,#262564,#262565,#262566,
#262567,#262568,#262569,#262570,#262571,#262572,#262573,#262574,#262575,
#262576,#262577,#262578,#262579,#262580,#262581,#262582,#262583,#262584,
#262585,#262586,#262587,#262588,#262589,#262590,#262591,#262592,#262593,
#262594,#262595,#262596,#262597,#262598,#262599,#262600,#262601,#262602,
#262603,#262604,#262605,#262606,#262607,#262608,#262609,#262610,#262611,
#262612,#262613,#262614,#262615,#262616,#262617,#262618,#262619,#262620,
#262621,#262622,#262623,#262624,#262625,#262626,#262627,#262628,#262629,
#262630,#262631,#262632,#262633,#262634,#262635,#262636,#262637,#262638,
#262639,#262640,#262641,#262642,#262643,#262644,#262645,#262646,#262647,
#262648,#262649),(#262650,#262651,#262652,#262653,#262654,#262655,#262656,
#262657,#262658,#262659,#262660,#262661,#262662,#262663,#262664,#262665,
#262666,#262667,#262668,#262669,#262670,#262671,#262672,#262673,#262674,
#262675,#262676,#262677,#262678,#262679,#262680,#262681,#262682,#262683,
#262684,#262685,#262686,#262687,#262688,#262689,#262690,#262691,#262692,
#262693,#262694,#262695,#262696,#262697,#262698,#262699,#262700,#262701,
#262702,#262703,#262704,#262705,#262706,#262707,#262708,#262709,#262710,
#262711,#262712,#262713,#262714,#262715,#262716,#262717,#262718,#262719,
#262720,#262721,#262722,#262723,#262724,#262725,#262726,#262727,#262728,
#262729,#262730,#262731,#262732,#262733,#262734,#262735,#262736,#262737,
#262738,#262739,#262740,#262741,#262742,#262743,#262744,#262745,#262746,
#262747,#262748,#262749,#262750,#262751,#262752,#262753,#262754,#262755,
#262756,#262757,#262758,#262759,#262760,#262761,#262762,#262763,#262764,
#262765,#262766,#262767,#262768,#262769,#262770,#262771,#262772,#262773,
#262774,#262775,#262776,#262777,#262778,#262779,#262780,#262781,#262782,
#262783,#262784,#262785,#262786,#262787,#262788,#262789,#262790,#262791,
#262792,#262793,#262794,#262795,#262796,#262797,#262798,#262799,#262800,
#262801,#262802,#262803,#262804,#262805,#262806,#262807,#262808,#262809,
#262810)),.UNSPECIFIED.,.F.,.F.,.F.)
B_SPLINE_SURFACE_WITH_KNOTS((2,2),(3,2,2,2,2,2,2,2,2,2,2,2,2,2,2,2,2,2,
2,2,2,2,2,2,2,2,2,2,2,2,2,2,2,2,2,2,2,2,2,2,2,2,2,2,2,2,2,2,2,2,2,2,2,2,
2,2,2,2,2,2,2,2,2,2,2,2,2,2,2,2,2,2,2,2,2,2,2,2,2,2,3),(0.,1.),(0.,0.0125,
0.025,0.0375,0.05,0.0625,0.075,0.0875,0.1,0.1125,0.125,0.1375,0.15,0.1625,
0.175,0.1875,0.2,0.2125,0.225,0.2375,0.25,0.2625,0.275,0.2875,0.3,0.3125,
0.325,0.3375,0.35,0.3625,0.375,0.3875,0.4,0.4125,0.425,0.4375,0.45,0.4625,
0.475,0.4875,0.5,0.5125,0.525,0.5375,0.55,0.5625,0.575,0.5875,0.6,0.6125,
0.625,0.6375,0.65,0.6625,0.675,0.6875,0.7,0.7125,0.725,0.7375,0.75,0.7625,
0.775,0.7875,0.8,0.8125,0.825,0.8375,0.85,0.8625,0.875,0.8875,0.9,0.9125,
0.925,0.9375,0.95,0.9625,0.975,0.9875,1.),.UNSPECIFIED.)
GEOMETRIC_REPRESENTATION_ITEM()
RATIONAL_B_SPLINE_SURFACE(((1.,0.923879532511287,1.,0.923879532511287,1.,
0.923879532511287,1.,0.923879532511287,1.,0.923879532511287,1.,0.923879532511287,
1.,0.923879532511287,1.,0.923879532511287,1.,0.923879532511287,1.,0.923879532511287,
1.,0.923879532511287,1.,0.923879532511287,1.,0.923879532511287,1.,0.923879532511287,
1.,0.923879532511287,1.,0.923879532511287,1.,0.923879532511287,1.,0.923879532511287,
1.,0.923879532511287,1.,0.923879532511287,1.,0.923879532511287,1.,0.923879532511287,
1.,0.923879532511287,1.,0.923879532511287,1.,0.923879532511287,1.,0.923879532511287,
1.,0.923879532511287,1.,0.923879532511287,1.,0.923879532511287,1.,0.923879532511287,
1.,0.923879532511287,1.,0.923879532511287,1.,0.923879532511287,1.,0.923879532511287,
1.,0.923879532511287,1.,0.923879532511287,1.,0.923879532511287,1.,0.923879532511287,
1.,0.923879532511287,1.,0.923879532511287,1.,0.923879532511287,1.,0.923879532511287,
1.,0.923879532511287,1.,0.923879532511287,1.,0.923879532511287,1.,0.923879532511287,
1.,0.923879532511287,1.,0.923879532511287,1.,0.923879532511287,1.,0.923879532511287,
1.,0.923879532511287,1.,0.923879532511287,1.,0.923879532511287,1.,0.923879532511287,
1.,0.923879532511287,1.,0.923879532511287,1.,0.923879532511287,1.,0.923879532511287,
1.,0.923879532511287,1.,0.923879532511287,1.,0.923879532511287,1.,0.923879532511287,
1.,0.923879532511287,1.,0.923879532511287,1.,0.923879532511287,1.,0.923879532511287,
1.,0.923879532511287,1.,0.923879532511287,1.,0.923879532511287,1.,0.923879532511287,
1.,0.923879532511287,1.,0.923879532511287,1.,0.923879532511287,1.,0.923879532511287,
1.,0.923879532511287,1.,0.923879532511287,1.,0.923879532511287,1.,0.923879532511287,
1.,0.923879532511287,1.,0.923879532511287,1.),(1.,0.923879532511287,1.,
0.923879532511287,1.,0.923879532511287,1.,0.923879532511287,1.,0.923879532511287,
1.,0.923879532511287,1.,0.923879532511287,1.,0.923879532511287,1.,0.923879532511287,
1.,0.923879532511287,1.,0.923879532511287,1.,0.923879532511287,1.,0.923879532511287,
1.,0.923879532511287,1.,0.923879532511287,1.,0.923879532511287,1.,0.923879532511287,
1.,0.923879532511287,1.,0.923879532511287,1.,0.923879532511287,1.,0.923879532511287,
1.,0.923879532511287,1.,0.923879532511287,1.,0.923879532511287,1.,0.923879532511287,
1.,0.923879532511287,1.,0.923879532511287,1.,0.923879532511287,1.,0.923879532511287,
1.,0.923879532511287,1.,0.923879532511287,1.,0.923879532511287,1.,0.923879532511287,
1.,0.923879532511287,1.,0.923879532511287,1.,0.923879532511287,1.,0.923879532511287,
1.,0.923879532511287,1.,0.923879532511287,1.,0.923879532511287,1.,0.923879532511287,
1.,0.923879532511287,1.,0.923879532511287,1.,0.923879532511287,1.,0.923879532511287,
1.,0.923879532511287,1.,0.923879532511287,1.,0.923879532511287,1.,0.923879532511287,
1.,0.923879532511287,1.,0.923879532511287,1.,0.923879532511287,1.,0.923879532511287,
1.,0.923879532511287,1.,0.923879532511287,1.,0.923879532511287,1.,0.923879532511287,
1.,0.923879532511287,1.,0.923879532511287,1.,0.923879532511287,1.,0.923879532511287,
1.,0.923879532511287,1.,0.923879532511287,1.,0.923879532511287,1.,0.923879532511287,
1.,0.923879532511287,1.,0.923879532511287,1.,0.923879532511287,1.,0.923879532511287,
1.,0.923879532511287,1.,0.923879532511287,1.,0.923879532511287,1.,0.923879532511287,
1.,0.923879532511287,1.,0.923879532511287,1.,0.923879532511287,1.,0.923879532511287,
1.,0.923879532511287,1.,0.923879532511287,1.,0.923879532511287,1.)))
REPRESENTATION_ITEM('')
SURFACE()
);
#4014=(
BOUNDED_SURFACE()
B_SPLINE_SURFACE(1,2,((#262846,#262847,#262848,#262849,#262850,#262851,
#262852,#262853,#262854,#262855,#262856,#262857,#262858,#262859,#262860,
#262861,#262862,#262863,#262864,#262865,#262866,#262867,#262868,#262869,
#262870,#262871,#262872,#262873,#262874,#262875,#262876,#262877,#262878,
#262879,#262880,#262881,#262882,#262883,#262884,#262885,#262886,#262887,
#262888,#262889,#262890,#262891,#262892,#262893,#262894,#262895,#262896,
#262897,#262898,#262899,#262900,#262901,#262902,#262903,#262904,#262905,
#262906,#262907,#262908,#262909,#262910,#262911,#262912,#262913,#262914,
#262915,#262916,#262917,#262918,#262919,#262920,#262921,#262922,#262923,
#262924,#262925,#262926,#262927,#262928,#262929,#262930,#262931,#262932,
#262933,#262934,#262935,#262936,#262937,#262938,#262939,#262940,#262941,
#262942,#262943,#262944,#262945,#262946,#262947,#262948,#262949,#262950,
#262951,#262952,#262953,#262954,#262955,#262956,#262957,#262958,#262959,
#262960,#262961,#262962,#262963,#262964,#262965,#262966,#262967,#262968,
#262969,#262970,#262971,#262972,#262973,#262974,#262975,#262976,#262977,
#262978,#262979,#262980,#262981,#262982,#262983,#262984,#262985,#262986,
#262987,#262988,#262989,#262990,#262991,#262992,#262993,#262994,#262995,
#262996,#262997,#262998,#262999,#263000,#263001,#263002,#263003,#263004,
#263005,#263006),(#263007,#263008,#263009,#263010,#263011,#263012,#263013,
#263014,#263015,#263016,#263017,#263018,#263019,#263020,#263021,#263022,
#263023,#263024,#263025,#263026,#263027,#263028,#263029,#263030,#263031,
#263032,#263033,#263034,#263035,#263036,#263037,#263038,#263039,#263040,
#263041,#263042,#263043,#263044,#263045,#263046,#263047,#263048,#263049,
#263050,#263051,#263052,#263053,#263054,#263055,#263056,#263057,#263058,
#263059,#263060,#263061,#263062,#263063,#263064,#263065,#263066,#263067,
#263068,#263069,#263070,#263071,#263072,#263073,#263074,#263075,#263076,
#263077,#263078,#263079,#263080,#263081,#263082,#263083,#263084,#263085,
#263086,#263087,#263088,#263089,#263090,#263091,#263092,#263093,#263094,
#263095,#263096,#263097,#263098,#263099,#263100,#263101,#263102,#263103,
#263104,#263105,#263106,#263107,#263108,#263109,#263110,#263111,#263112,
#263113,#263114,#263115,#263116,#263117,#263118,#263119,#263120,#263121,
#263122,#263123,#263124,#263125,#263126,#263127,#263128,#263129,#263130,
#263131,#263132,#263133,#263134,#263135,#263136,#263137,#263138,#263139,
#263140,#263141,#263142,#263143,#263144,#263145,#263146,#263147,#263148,
#263149,#263150,#263151,#263152,#263153,#263154,#263155,#263156,#263157,
#263158,#263159,#263160,#263161,#263162,#263163,#263164,#263165,#263166,
#263167)),.UNSPECIFIED.,.F.,.F.,.F.)
B_SPLINE_SURFACE_WITH_KNOTS((2,2),(3,2,2,2,2,2,2,2,2,2,2,2,2,2,2,2,2,2,
2,2,2,2,2,2,2,2,2,2,2,2,2,2,2,2,2,2,2,2,2,2,2,2,2,2,2,2,2,2,2,2,2,2,2,2,
2,2,2,2,2,2,2,2,2,2,2,2,2,2,2,2,2,2,2,2,2,2,2,2,2,2,3),(0.,1.),(0.,0.0125,
0.025,0.0375,0.05,0.0625,0.075,0.0875,0.1,0.1125,0.125,0.1375,0.15,0.1625,
0.175,0.1875,0.2,0.2125,0.225,0.2375,0.25,0.2625,0.275,0.2875,0.3,0.3125,
0.325,0.3375,0.35,0.3625,0.375,0.3875,0.4,0.4125,0.425,0.4375,0.45,0.4625,
0.475,0.4875,0.5,0.5125,0.525,0.5375,0.55,0.5625,0.575,0.5875,0.6,0.6125,
0.625,0.6375,0.65,0.6625,0.675,0.6875,0.7,0.7125,0.725,0.7375,0.75,0.7625,
0.775,0.7875,0.8,0.8125,0.825,0.8375,0.85,0.8625,0.875,0.8875,0.9,0.9125,
0.925,0.9375,0.95,0.9625,0.975,0.9875,1.),.UNSPECIFIED.)
GEOMETRIC_REPRESENTATION_ITEM()
RATIONAL_B_SPLINE_SURFACE(((1.,0.923879532511287,1.,0.923879532511287,1.,
0.923879532511287,1.,0.923879532511287,1.,0.923879532511287,1.,0.923879532511287,
1.,0.923879532511287,1.,0.923879532511287,1.,0.923879532511287,1.,0.923879532511287,
1.,0.923879532511287,1.,0.923879532511287,1.,0.923879532511287,1.,0.923879532511287,
1.,0.923879532511287,1.,0.923879532511287,1.,0.923879532511287,1.,0.923879532511287,
1.,0.923879532511287,1.,0.923879532511287,1.,0.923879532511287,1.,0.923879532511287,
1.,0.923879532511287,1.,0.923879532511287,1.,0.923879532511287,1.,0.923879532511287,
1.,0.923879532511287,1.,0.923879532511287,1.,0.923879532511287,1.,0.923879532511287,
1.,0.923879532511287,1.,0.923879532511287,1.,0.923879532511287,1.,0.923879532511287,
1.,0.923879532511287,1.,0.923879532511287,1.,0.923879532511287,1.,0.923879532511287,
1.,0.923879532511287,1.,0.923879532511287,1.,0.923879532511287,1.,0.923879532511287,
1.,0.923879532511287,1.,0.923879532511287,1.,0.923879532511287,1.,0.923879532511287,
1.,0.923879532511287,1.,0.923879532511287,1.,0.923879532511287,1.,0.923879532511287,
1.,0.923879532511287,1.,0.923879532511287,1.,0.923879532511287,1.,0.923879532511287,
1.,0.923879532511287,1.,0.923879532511287,1.,0.923879532511287,1.,0.923879532511287,
1.,0.923879532511287,1.,0.923879532511287,1.,0.923879532511287,1.,0.923879532511287,
1.,0.923879532511287,1.,0.923879532511287,1.,0.923879532511287,1.,0.923879532511287,
1.,0.923879532511287,1.,0.923879532511287,1.,0.923879532511287,1.,0.923879532511287,
1.,0.923879532511287,1.,0.923879532511287,1.,0.923879532511287,1.,0.923879532511287,
1.,0.923879532511287,1.,0.923879532511287,1.,0.923879532511287,1.,0.923879532511287,
1.,0.923879532511287,1.,0.923879532511287,1.),(1.,0.923879532511287,1.,
0.923879532511287,1.,0.923879532511287,1.,0.923879532511287,1.,0.923879532511287,
1.,0.923879532511287,1.,0.923879532511287,1.,0.923879532511287,1.,0.923879532511287,
1.,0.923879532511287,1.,0.923879532511287,1.,0.923879532511287,1.,0.923879532511287,
1.,0.923879532511287,1.,0.923879532511287,1.,0.923879532511287,1.,0.923879532511287,
1.,0.923879532511287,1.,0.923879532511287,1.,0.923879532511287,1.,0.923879532511287,
1.,0.923879532511287,1.,0.923879532511287,1.,0.923879532511287,1.,0.923879532511287,
1.,0.923879532511287,1.,0.923879532511287,1.,0.923879532511287,1.,0.923879532511287,
1.,0.923879532511287,1.,0.923879532511287,1.,0.923879532511287,1.,0.923879532511287,
1.,0.923879532511287,1.,0.923879532511287,1.,0.923879532511287,1.,0.923879532511287,
1.,0.923879532511287,1.,0.923879532511287,1.,0.923879532511287,1.,0.923879532511287,
1.,0.923879532511287,1.,0.923879532511287,1.,0.923879532511287,1.,0.923879532511287,
1.,0.923879532511287,1.,0.923879532511287,1.,0.923879532511287,1.,0.923879532511287,
1.,0.923879532511287,1.,0.923879532511287,1.,0.923879532511287,1.,0.923879532511287,
1.,0.923879532511287,1.,0.923879532511287,1.,0.923879532511287,1.,0.923879532511287,
1.,0.923879532511287,1.,0.923879532511287,1.,0.923879532511287,1.,0.923879532511287,
1.,0.923879532511287,1.,0.923879532511287,1.,0.923879532511287,1.,0.923879532511287,
1.,0.923879532511287,1.,0.923879532511287,1.,0.923879532511287,1.,0.923879532511287,
1.,0.923879532511287,1.,0.923879532511287,1.,0.923879532511287,1.,0.923879532511287,
1.,0.923879532511287,1.,0.923879532511287,1.,0.923879532511287,1.,0.923879532511287,
1.,0.923879532511287,1.,0.923879532511287,1.,0.923879532511287,1.)))
REPRESENTATION_ITEM('')
SURFACE()
);
#4015=(
BOUNDED_SURFACE()
B_SPLINE_SURFACE(1,2,((#264016,#264017,#264018,#264019,#264020,#264021,
#264022,#264023,#264024,#264025,#264026,#264027,#264028,#264029,#264030,
#264031,#264032,#264033,#264034,#264035,#264036,#264037,#264038,#264039,
#264040,#264041,#264042,#264043,#264044,#264045,#264046,#264047,#264048,
#264049,#264050,#264051,#264052,#264053,#264054,#264055,#264056,#264057,
#264058,#264059,#264060,#264061,#264062,#264063,#264064,#264065,#264066,
#264067,#264068,#264069,#264070,#264071,#264072,#264073,#264074,#264075,
#264076,#264077,#264078,#264079,#264080,#264081,#264082,#264083,#264084,
#264085,#264086,#264087,#264088,#264089,#264090,#264091,#264092,#264093,
#264094,#264095,#264096,#264097,#264098,#264099,#264100,#264101,#264102,
#264103,#264104,#264105,#264106,#264107,#264108,#264109,#264110,#264111,
#264112,#264113,#264114,#264115,#264116,#264117,#264118,#264119,#264120,
#264121,#264122,#264123,#264124,#264125,#264126,#264127,#264128,#264129,
#264130,#264131,#264132,#264133,#264134,#264135,#264136,#264137,#264138,
#264139,#264140,#264141,#264142,#264143,#264144,#264145,#264146,#264147,
#264148,#264149,#264150,#264151,#264152,#264153,#264154,#264155,#264156,
#264157,#264158,#264159,#264160,#264161,#264162,#264163,#264164,#264165,
#264166,#264167,#264168,#264169,#264170,#264171,#264172,#264173,#264174,
#264175,#264176),(#264177,#264178,#264179,#264180,#264181,#264182,#264183,
#264184,#264185,#264186,#264187,#264188,#264189,#264190,#264191,#264192,
#264193,#264194,#264195,#264196,#264197,#264198,#264199,#264200,#264201,
#264202,#264203,#264204,#264205,#264206,#264207,#264208,#264209,#264210,
#264211,#264212,#264213,#264214,#264215,#264216,#264217,#264218,#264219,
#264220,#264221,#264222,#264223,#264224,#264225,#264226,#264227,#264228,
#264229,#264230,#264231,#264232,#264233,#264234,#264235,#264236,#264237,
#264238,#264239,#264240,#264241,#264242,#264243,#264244,#264245,#264246,
#264247,#264248,#264249,#264250,#264251,#264252,#264253,#264254,#264255,
#264256,#264257,#264258,#264259,#264260,#264261,#264262,#264263,#264264,
#264265,#264266,#264267,#264268,#264269,#264270,#264271,#264272,#264273,
#264274,#264275,#264276,#264277,#264278,#264279,#264280,#264281,#264282,
#264283,#264284,#264285,#264286,#264287,#264288,#264289,#264290,#264291,
#264292,#264293,#264294,#264295,#264296,#264297,#264298,#264299,#264300,
#264301,#264302,#264303,#264304,#264305,#264306,#264307,#264308,#264309,
#264310,#264311,#264312,#264313,#264314,#264315,#264316,#264317,#264318,
#264319,#264320,#264321,#264322,#264323,#264324,#264325,#264326,#264327,
#264328,#264329,#264330,#264331,#264332,#264333,#264334,#264335,#264336,
#264337)),.UNSPECIFIED.,.F.,.F.,.F.)
B_SPLINE_SURFACE_WITH_KNOTS((2,2),(3,2,2,2,2,2,2,2,2,2,2,2,2,2,2,2,2,2,
2,2,2,2,2,2,2,2,2,2,2,2,2,2,2,2,2,2,2,2,2,2,2,2,2,2,2,2,2,2,2,2,2,2,2,2,
2,2,2,2,2,2,2,2,2,2,2,2,2,2,2,2,2,2,2,2,2,2,2,2,2,2,3),(0.,1.),(0.,0.0125,
0.025,0.0375,0.05,0.0625,0.075,0.0875,0.1,0.1125,0.125,0.1375,0.15,0.1625,
0.175,0.1875,0.2,0.2125,0.225,0.2375,0.25,0.2625,0.275,0.2875,0.3,0.3125,
0.325,0.3375,0.35,0.3625,0.375,0.3875,0.4,0.4125,0.425,0.4375,0.45,0.4625,
0.475,0.4875,0.5,0.5125,0.525,0.5375,0.55,0.5625,0.575,0.5875,0.6,0.6125,
0.625,0.6375,0.65,0.6625,0.675,0.6875,0.7,0.7125,0.725,0.7375,0.75,0.7625,
0.775,0.7875,0.8,0.8125,0.825,0.8375,0.85,0.8625,0.875,0.8875,0.9,0.9125,
0.925,0.9375,0.95,0.9625,0.975,0.9875,1.),.UNSPECIFIED.)
GEOMETRIC_REPRESENTATION_ITEM()
RATIONAL_B_SPLINE_SURFACE(((1.,0.923879532511287,1.,0.923879532511287,1.,
0.923879532511287,1.,0.923879532511287,1.,0.923879532511287,1.,0.923879532511287,
1.,0.923879532511287,1.,0.923879532511287,1.,0.923879532511287,1.,0.923879532511287,
1.,0.923879532511287,1.,0.923879532511287,1.,0.923879532511287,1.,0.923879532511287,
1.,0.923879532511287,1.,0.923879532511287,1.,0.923879532511287,1.,0.923879532511287,
1.,0.923879532511287,1.,0.923879532511287,1.,0.923879532511287,1.,0.923879532511287,
1.,0.923879532511287,1.,0.923879532511287,1.,0.923879532511287,1.,0.923879532511287,
1.,0.923879532511287,1.,0.923879532511287,1.,0.923879532511287,1.,0.923879532511287,
1.,0.923879532511287,1.,0.923879532511287,1.,0.923879532511287,1.,0.923879532511287,
1.,0.923879532511287,1.,0.923879532511287,1.,0.923879532511287,1.,0.923879532511287,
1.,0.923879532511287,1.,0.923879532511287,1.,0.923879532511287,1.,0.923879532511287,
1.,0.923879532511287,1.,0.923879532511287,1.,0.923879532511287,1.,0.923879532511287,
1.,0.923879532511287,1.,0.923879532511287,1.,0.923879532511287,1.,0.923879532511287,
1.,0.923879532511287,1.,0.923879532511287,1.,0.923879532511287,1.,0.923879532511287,
1.,0.923879532511287,1.,0.923879532511287,1.,0.923879532511287,1.,0.923879532511287,
1.,0.923879532511287,1.,0.923879532511287,1.,0.923879532511287,1.,0.923879532511287,
1.,0.923879532511287,1.,0.923879532511287,1.,0.923879532511287,1.,0.923879532511287,
1.,0.923879532511287,1.,0.923879532511287,1.,0.923879532511287,1.,0.923879532511287,
1.,0.923879532511287,1.,0.923879532511287,1.,0.923879532511287,1.,0.923879532511287,
1.,0.923879532511287,1.,0.923879532511287,1.,0.923879532511287,1.,0.923879532511287,
1.,0.923879532511287,1.,0.923879532511287,1.),(1.,0.923879532511287,1.,
0.923879532511287,1.,0.923879532511287,1.,0.923879532511287,1.,0.923879532511287,
1.,0.923879532511287,1.,0.923879532511287,1.,0.923879532511287,1.,0.923879532511287,
1.,0.923879532511287,1.,0.923879532511287,1.,0.923879532511287,1.,0.923879532511287,
1.,0.923879532511287,1.,0.923879532511287,1.,0.923879532511287,1.,0.923879532511287,
1.,0.923879532511287,1.,0.923879532511287,1.,0.923879532511287,1.,0.923879532511287,
1.,0.923879532511287,1.,0.923879532511287,1.,0.923879532511287,1.,0.923879532511287,
1.,0.923879532511287,1.,0.923879532511287,1.,0.923879532511287,1.,0.923879532511287,
1.,0.923879532511287,1.,0.923879532511287,1.,0.923879532511287,1.,0.923879532511287,
1.,0.923879532511287,1.,0.923879532511287,1.,0.923879532511287,1.,0.923879532511287,
1.,0.923879532511287,1.,0.923879532511287,1.,0.923879532511287,1.,0.923879532511287,
1.,0.923879532511287,1.,0.923879532511287,1.,0.923879532511287,1.,0.923879532511287,
1.,0.923879532511287,1.,0.923879532511287,1.,0.923879532511287,1.,0.923879532511287,
1.,0.923879532511287,1.,0.923879532511287,1.,0.923879532511287,1.,0.923879532511287,
1.,0.923879532511287,1.,0.923879532511287,1.,0.923879532511287,1.,0.923879532511287,
1.,0.923879532511287,1.,0.923879532511287,1.,0.923879532511287,1.,0.923879532511287,
1.,0.923879532511287,1.,0.923879532511287,1.,0.923879532511287,1.,0.923879532511287,
1.,0.923879532511287,1.,0.923879532511287,1.,0.923879532511287,1.,0.923879532511287,
1.,0.923879532511287,1.,0.923879532511287,1.,0.923879532511287,1.,0.923879532511287,
1.,0.923879532511287,1.,0.923879532511287,1.,0.923879532511287,1.,0.923879532511287,
1.,0.923879532511287,1.,0.923879532511287,1.,0.923879532511287,1.)))
REPRESENTATION_ITEM('')
SURFACE()
);
#4016=(
BOUNDED_SURFACE()
B_SPLINE_SURFACE(1,2,((#264373,#264374,#264375,#264376,#264377,#264378,
#264379,#264380,#264381,#264382,#264383,#264384,#264385,#264386,#264387,
#264388,#264389,#264390,#264391,#264392,#264393,#264394,#264395,#264396,
#264397,#264398,#264399,#264400,#264401,#264402,#264403,#264404,#264405,
#264406,#264407,#264408,#264409,#264410,#264411,#264412,#264413,#264414,
#264415,#264416,#264417,#264418,#264419,#264420,#264421,#264422,#264423,
#264424,#264425,#264426,#264427,#264428,#264429,#264430,#264431,#264432,
#264433,#264434,#264435,#264436,#264437,#264438,#264439,#264440,#264441,
#264442,#264443,#264444,#264445,#264446,#264447,#264448,#264449,#264450,
#264451,#264452,#264453,#264454,#264455,#264456,#264457,#264458,#264459,
#264460,#264461,#264462,#264463,#264464,#264465,#264466,#264467,#264468,
#264469,#264470,#264471,#264472,#264473,#264474,#264475,#264476,#264477,
#264478,#264479,#264480,#264481,#264482,#264483,#264484,#264485,#264486,
#264487,#264488,#264489,#264490,#264491,#264492,#264493,#264494,#264495,
#264496,#264497,#264498,#264499,#264500,#264501,#264502,#264503,#264504,
#264505,#264506,#264507,#264508,#264509,#264510,#264511,#264512,#264513,
#264514,#264515,#264516,#264517,#264518,#264519,#264520,#264521,#264522,
#264523,#264524,#264525,#264526,#264527,#264528,#264529,#264530,#264531,
#264532,#264533),(#264534,#264535,#264536,#264537,#264538,#264539,#264540,
#264541,#264542,#264543,#264544,#264545,#264546,#264547,#264548,#264549,
#264550,#264551,#264552,#264553,#264554,#264555,#264556,#264557,#264558,
#264559,#264560,#264561,#264562,#264563,#264564,#264565,#264566,#264567,
#264568,#264569,#264570,#264571,#264572,#264573,#264574,#264575,#264576,
#264577,#264578,#264579,#264580,#264581,#264582,#264583,#264584,#264585,
#264586,#264587,#264588,#264589,#264590,#264591,#264592,#264593,#264594,
#264595,#264596,#264597,#264598,#264599,#264600,#264601,#264602,#264603,
#264604,#264605,#264606,#264607,#264608,#264609,#264610,#264611,#264612,
#264613,#264614,#264615,#264616,#264617,#264618,#264619,#264620,#264621,
#264622,#264623,#264624,#264625,#264626,#264627,#264628,#264629,#264630,
#264631,#264632,#264633,#264634,#264635,#264636,#264637,#264638,#264639,
#264640,#264641,#264642,#264643,#264644,#264645,#264646,#264647,#264648,
#264649,#264650,#264651,#264652,#264653,#264654,#264655,#264656,#264657,
#264658,#264659,#264660,#264661,#264662,#264663,#264664,#264665,#264666,
#264667,#264668,#264669,#264670,#264671,#264672,#264673,#264674,#264675,
#264676,#264677,#264678,#264679,#264680,#264681,#264682,#264683,#264684,
#264685,#264686,#264687,#264688,#264689,#264690,#264691,#264692,#264693,
#264694)),.UNSPECIFIED.,.F.,.F.,.F.)
B_SPLINE_SURFACE_WITH_KNOTS((2,2),(3,2,2,2,2,2,2,2,2,2,2,2,2,2,2,2,2,2,
2,2,2,2,2,2,2,2,2,2,2,2,2,2,2,2,2,2,2,2,2,2,2,2,2,2,2,2,2,2,2,2,2,2,2,2,
2,2,2,2,2,2,2,2,2,2,2,2,2,2,2,2,2,2,2,2,2,2,2,2,2,2,3),(0.,1.),(0.,0.0125,
0.025,0.0375,0.05,0.0625,0.075,0.0875,0.1,0.1125,0.125,0.1375,0.15,0.1625,
0.175,0.1875,0.2,0.2125,0.225,0.2375,0.25,0.2625,0.275,0.2875,0.3,0.3125,
0.325,0.3375,0.35,0.3625,0.375,0.3875,0.4,0.4125,0.425,0.4375,0.45,0.4625,
0.475,0.4875,0.5,0.5125,0.525,0.5375,0.55,0.5625,0.575,0.5875,0.6,0.6125,
0.625,0.6375,0.65,0.6625,0.675,0.6875,0.7,0.7125,0.725,0.7375,0.75,0.7625,
0.775,0.7875,0.8,0.8125,0.825,0.8375,0.85,0.8625,0.875,0.8875,0.9,0.9125,
0.925,0.9375,0.95,0.9625,0.975,0.9875,1.),.UNSPECIFIED.)
GEOMETRIC_REPRESENTATION_ITEM()
RATIONAL_B_SPLINE_SURFACE(((1.,0.923879532511287,1.,0.923879532511287,1.,
0.923879532511287,1.,0.923879532511287,1.,0.923879532511287,1.,0.923879532511287,
1.,0.923879532511287,1.,0.923879532511287,1.,0.923879532511287,1.,0.923879532511287,
1.,0.923879532511287,1.,0.923879532511287,1.,0.923879532511287,1.,0.923879532511287,
1.,0.923879532511287,1.,0.923879532511287,1.,0.923879532511287,1.,0.923879532511287,
1.,0.923879532511287,1.,0.923879532511287,1.,0.923879532511287,1.,0.923879532511287,
1.,0.923879532511287,1.,0.923879532511287,1.,0.923879532511287,1.,0.923879532511287,
1.,0.923879532511287,1.,0.923879532511287,1.,0.923879532511287,1.,0.923879532511287,
1.,0.923879532511287,1.,0.923879532511287,1.,0.923879532511287,1.,0.923879532511287,
1.,0.923879532511287,1.,0.923879532511287,1.,0.923879532511287,1.,0.923879532511287,
1.,0.923879532511287,1.,0.923879532511287,1.,0.923879532511287,1.,0.923879532511287,
1.,0.923879532511287,1.,0.923879532511287,1.,0.923879532511287,1.,0.923879532511287,
1.,0.923879532511287,1.,0.923879532511287,1.,0.923879532511287,1.,0.923879532511287,
1.,0.923879532511287,1.,0.923879532511287,1.,0.923879532511287,1.,0.923879532511287,
1.,0.923879532511287,1.,0.923879532511287,1.,0.923879532511287,1.,0.923879532511287,
1.,0.923879532511287,1.,0.923879532511287,1.,0.923879532511287,1.,0.923879532511287,
1.,0.923879532511287,1.,0.923879532511287,1.,0.923879532511287,1.,0.923879532511287,
1.,0.923879532511287,1.,0.923879532511287,1.,0.923879532511287,1.,0.923879532511287,
1.,0.923879532511287,1.,0.923879532511287,1.,0.923879532511287,1.,0.923879532511287,
1.,0.923879532511287,1.,0.923879532511287,1.,0.923879532511287,1.,0.923879532511287,
1.,0.923879532511287,1.,0.923879532511287,1.),(1.,0.923879532511287,1.,
0.923879532511287,1.,0.923879532511287,1.,0.923879532511287,1.,0.923879532511287,
1.,0.923879532511287,1.,0.923879532511287,1.,0.923879532511287,1.,0.923879532511287,
1.,0.923879532511287,1.,0.923879532511287,1.,0.923879532511287,1.,0.923879532511287,
1.,0.923879532511287,1.,0.923879532511287,1.,0.923879532511287,1.,0.923879532511287,
1.,0.923879532511287,1.,0.923879532511287,1.,0.923879532511287,1.,0.923879532511287,
1.,0.923879532511287,1.,0.923879532511287,1.,0.923879532511287,1.,0.923879532511287,
1.,0.923879532511287,1.,0.923879532511287,1.,0.923879532511287,1.,0.923879532511287,
1.,0.923879532511287,1.,0.923879532511287,1.,0.923879532511287,1.,0.923879532511287,
1.,0.923879532511287,1.,0.923879532511287,1.,0.923879532511287,1.,0.923879532511287,
1.,0.923879532511287,1.,0.923879532511287,1.,0.923879532511287,1.,0.923879532511287,
1.,0.923879532511287,1.,0.923879532511287,1.,0.923879532511287,1.,0.923879532511287,
1.,0.923879532511287,1.,0.923879532511287,1.,0.923879532511287,1.,0.923879532511287,
1.,0.923879532511287,1.,0.923879532511287,1.,0.923879532511287,1.,0.923879532511287,
1.,0.923879532511287,1.,0.923879532511287,1.,0.923879532511287,1.,0.923879532511287,
1.,0.923879532511287,1.,0.923879532511287,1.,0.923879532511287,1.,0.923879532511287,
1.,0.923879532511287,1.,0.923879532511287,1.,0.923879532511287,1.,0.923879532511287,
1.,0.923879532511287,1.,0.923879532511287,1.,0.923879532511287,1.,0.923879532511287,
1.,0.923879532511287,1.,0.923879532511287,1.,0.923879532511287,1.,0.923879532511287,
1.,0.923879532511287,1.,0.923879532511287,1.,0.923879532511287,1.,0.923879532511287,
1.,0.923879532511287,1.,0.923879532511287,1.,0.923879532511287,1.)))
REPRESENTATION_ITEM('')
SURFACE()
);
#4085=(
BOUNDED_CURVE()
B_SPLINE_CURVE(2,(#167184,#167185,#167186),.UNSPECIFIED.,.F.,.F.)
B_SPLINE_CURVE_WITH_KNOTS((3,3),(-1.90587960023829,-1.38751706971772),
 .UNSPECIFIED.)
CURVE()
GEOMETRIC_REPRESENTATION_ITEM()
RATIONAL_B_SPLINE_CURVE((1.66210638417239,1.76950594708369,1.76950594708369))
REPRESENTATION_ITEM('')
);
#4086=(
BOUNDED_CURVE()
B_SPLINE_CURVE(2,(#167187,#167188,#167189),.UNSPECIFIED.,.F.,.F.)
B_SPLINE_CURVE_WITH_KNOTS((3,3),(-1.38751706971772,-0.869154539197601),
 .UNSPECIFIED.)
CURVE()
GEOMETRIC_REPRESENTATION_ITEM()
RATIONAL_B_SPLINE_CURVE((1.7695059470837,1.7695059470837,1.66210638417259))
REPRESENTATION_ITEM('')
);
#4087=(
BOUNDED_CURVE()
B_SPLINE_CURVE(2,(#167201,#167202,#167203),.UNSPECIFIED.,.F.,.F.)
B_SPLINE_CURVE_WITH_KNOTS((3,3),(-1.90587960023829,-1.38751706971772),
 .UNSPECIFIED.)
CURVE()
GEOMETRIC_REPRESENTATION_ITEM()
RATIONAL_B_SPLINE_CURVE((1.66210638417239,1.76950594708369,1.76950594708369))
REPRESENTATION_ITEM('')
);
#4088=(
BOUNDED_CURVE()
B_SPLINE_CURVE(2,(#167216,#167217,#167218),.UNSPECIFIED.,.F.,.F.)
B_SPLINE_CURVE_WITH_KNOTS((3,3),(-1.38751706971771,-0.869154539197602),
 .UNSPECIFIED.)
CURVE()
GEOMETRIC_REPRESENTATION_ITEM()
RATIONAL_B_SPLINE_CURVE((1.76950594708369,1.76950594708369,1.66210638417258))
REPRESENTATION_ITEM('')
);
#4089=(
BOUNDED_CURVE()
B_SPLINE_CURVE(2,(#167259,#167260,#167261),.UNSPECIFIED.,.F.,.F.)
B_SPLINE_CURVE_WITH_KNOTS((3,3),(-1.9058796002383,-1.38751706971772),
 .UNSPECIFIED.)
CURVE()
GEOMETRIC_REPRESENTATION_ITEM()
RATIONAL_B_SPLINE_CURVE((1.66210638417238,1.76950594708369,1.76950594708369))
REPRESENTATION_ITEM('')
);
#4090=(
BOUNDED_CURVE()
B_SPLINE_CURVE(2,(#167262,#167263,#167264),.UNSPECIFIED.,.F.,.F.)
B_SPLINE_CURVE_WITH_KNOTS((3,3),(-1.38751706971773,-0.869154539197622),
 .UNSPECIFIED.)
CURVE()
GEOMETRIC_REPRESENTATION_ITEM()
RATIONAL_B_SPLINE_CURVE((1.76950594708368,1.76950594708368,1.66210638417257))
REPRESENTATION_ITEM('')
);
#4091=(
BOUNDED_CURVE()
B_SPLINE_CURVE(2,(#167267,#167268,#167269),.UNSPECIFIED.,.F.,.F.)
B_SPLINE_CURVE_WITH_KNOTS((3,3),(-1.90587960023789,-1.38751706971772),
 .UNSPECIFIED.)
CURVE()
GEOMETRIC_REPRESENTATION_ITEM()
RATIONAL_B_SPLINE_CURVE((1.66210638417255,1.76950594708369,1.76950594708369))
REPRESENTATION_ITEM('')
);
#4092=(
BOUNDED_CURVE()
B_SPLINE_CURVE(2,(#167281,#167282,#167283),.UNSPECIFIED.,.F.,.F.)
B_SPLINE_CURVE_WITH_KNOTS((3,3),(-1.38751706971772,-0.869154539197605),
 .UNSPECIFIED.)
CURVE()
GEOMETRIC_REPRESENTATION_ITEM()
RATIONAL_B_SPLINE_CURVE((1.76950594708369,1.76950594708369,1.66210638417258))
REPRESENTATION_ITEM('')
);
#4093=(
BOUNDED_CURVE()
B_SPLINE_CURVE(2,(#167286,#167287,#167288),.UNSPECIFIED.,.F.,.F.)
B_SPLINE_CURVE_WITH_KNOTS((3,3),(-1.90587960023829,-1.38751706971771),
 .UNSPECIFIED.)
CURVE()
GEOMETRIC_REPRESENTATION_ITEM()
RATIONAL_B_SPLINE_CURVE((1.66210638417239,1.76950594708369,1.76950594708369))
REPRESENTATION_ITEM('')
);
#4094=(
BOUNDED_CURVE()
B_SPLINE_CURVE(2,(#167300,#167301,#167302),.UNSPECIFIED.,.F.,.F.)
B_SPLINE_CURVE_WITH_KNOTS((3,3),(-1.38751706971772,-0.869154539197604),
 .UNSPECIFIED.)
CURVE()
GEOMETRIC_REPRESENTATION_ITEM()
RATIONAL_B_SPLINE_CURVE((1.76950594708369,1.76950594708369,1.66210638417258))
REPRESENTATION_ITEM('')
);
#4095=(
BOUNDED_CURVE()
B_SPLINE_CURVE(2,(#167305,#167306,#167307),.UNSPECIFIED.,.F.,.F.)
B_SPLINE_CURVE_WITH_KNOTS((3,3),(-1.90587960023783,-1.38751706971773),
 .UNSPECIFIED.)
CURVE()
GEOMETRIC_REPRESENTATION_ITEM()
RATIONAL_B_SPLINE_CURVE((1.66210638417257,1.76950594708368,1.76950594708368))
REPRESENTATION_ITEM('')
);
#4096=(
BOUNDED_CURVE()
B_SPLINE_CURVE(2,(#167319,#167320,#167321),.UNSPECIFIED.,.F.,.F.)
B_SPLINE_CURVE_WITH_KNOTS((3,3),(-1.38751706971772,-0.869154539197607),
 .UNSPECIFIED.)
CURVE()
GEOMETRIC_REPRESENTATION_ITEM()
RATIONAL_B_SPLINE_CURVE((1.76950594708369,1.76950594708369,1.66210638417258))
REPRESENTATION_ITEM('')
);
#4097=(
BOUNDED_CURVE()
B_SPLINE_CURVE(2,(#167324,#167325,#167326),.UNSPECIFIED.,.F.,.F.)
B_SPLINE_CURVE_WITH_KNOTS((3,3),(-1.90587960023828,-1.38751706971773),
 .UNSPECIFIED.)
CURVE()
GEOMETRIC_REPRESENTATION_ITEM()
RATIONAL_B_SPLINE_CURVE((1.66210638417238,1.76950594708368,1.76950594708368))
REPRESENTATION_ITEM('')
);
#4098=(
BOUNDED_CURVE()
B_SPLINE_CURVE(2,(#167338,#167339,#167340),.UNSPECIFIED.,.F.,.F.)
B_SPLINE_CURVE_WITH_KNOTS((3,3),(-1.38751706971773,-0.869154539197555),
 .UNSPECIFIED.)
CURVE()
GEOMETRIC_REPRESENTATION_ITEM()
RATIONAL_B_SPLINE_CURVE((1.76950594708368,1.76950594708368,1.66210638417254))
REPRESENTATION_ITEM('')
);
#4099=(
BOUNDED_CURVE()
B_SPLINE_CURVE(2,(#167354,#167355,#167356),.UNSPECIFIED.,.F.,.F.)
B_SPLINE_CURVE_WITH_KNOTS((3,3),(-1.90587960023789,-1.38751706971771),
 .UNSPECIFIED.)
CURVE()
GEOMETRIC_REPRESENTATION_ITEM()
RATIONAL_B_SPLINE_CURVE((1.66210638417255,1.7695059470837,1.7695059470837))
REPRESENTATION_ITEM('')
);
#4100=(
BOUNDED_CURVE()
B_SPLINE_CURVE(2,(#167368,#167369,#167370),.UNSPECIFIED.,.F.,.F.)
B_SPLINE_CURVE_WITH_KNOTS((3,3),(-1.38751706971771,-0.869154539197607),
 .UNSPECIFIED.)
CURVE()
GEOMETRIC_REPRESENTATION_ITEM()
RATIONAL_B_SPLINE_CURVE((1.7695059470837,1.7695059470837,1.66210638417258))
REPRESENTATION_ITEM('')
);
#4101=(
BOUNDED_CURVE()
B_SPLINE_CURVE(2,(#167373,#167374,#167375),.UNSPECIFIED.,.F.,.F.)
B_SPLINE_CURVE_WITH_KNOTS((3,3),(-1.90587960023829,-1.38751706971771),
 .UNSPECIFIED.)
CURVE()
GEOMETRIC_REPRESENTATION_ITEM()
RATIONAL_B_SPLINE_CURVE((1.66210638417239,1.76950594708369,1.76950594708369))
REPRESENTATION_ITEM('')
);
#4102=(
BOUNDED_CURVE()
B_SPLINE_CURVE(2,(#167387,#167388,#167389),.UNSPECIFIED.,.F.,.F.)
B_SPLINE_CURVE_WITH_KNOTS((3,3),(-1.38751706971771,-0.869154539197605),
 .UNSPECIFIED.)
CURVE()
GEOMETRIC_REPRESENTATION_ITEM()
RATIONAL_B_SPLINE_CURVE((1.7695059470837,1.76950594708369,1.66210638417258))
REPRESENTATION_ITEM('')
);
#4103=(
BOUNDED_CURVE()
B_SPLINE_CURVE(2,(#167392,#167393,#167394),.UNSPECIFIED.,.F.,.F.)
B_SPLINE_CURVE_WITH_KNOTS((3,3),(-1.90587960023829,-1.38751706971772),
 .UNSPECIFIED.)
CURVE()
GEOMETRIC_REPRESENTATION_ITEM()
RATIONAL_B_SPLINE_CURVE((1.66210638417239,1.7695059470837,1.7695059470837))
REPRESENTATION_ITEM('')
);
#4104=(
BOUNDED_CURVE()
B_SPLINE_CURVE(2,(#167406,#167407,#167408),.UNSPECIFIED.,.F.,.F.)
B_SPLINE_CURVE_WITH_KNOTS((3,3),(-1.38751706971771,-0.869154539197604),
 .UNSPECIFIED.)
CURVE()
GEOMETRIC_REPRESENTATION_ITEM()
RATIONAL_B_SPLINE_CURVE((1.76950594708369,1.76950594708369,1.66210638417258))
REPRESENTATION_ITEM('')
);
#4105=(
BOUNDED_CURVE()
B_SPLINE_CURVE(2,(#167411,#167412,#167413),.UNSPECIFIED.,.F.,.F.)
B_SPLINE_CURVE_WITH_KNOTS((3,3),(-1.90587960023783,-1.38751706971772),
 .UNSPECIFIED.)
CURVE()
GEOMETRIC_REPRESENTATION_ITEM()
RATIONAL_B_SPLINE_CURVE((1.66210638417258,1.7695059470837,1.7695059470837))
REPRESENTATION_ITEM('')
);
#4106=(
BOUNDED_CURVE()
B_SPLINE_CURVE(2,(#167425,#167426,#167427),.UNSPECIFIED.,.F.,.F.)
B_SPLINE_CURVE_WITH_KNOTS((3,3),(-1.38751706971772,-0.869154539197609),
 .UNSPECIFIED.)
CURVE()
GEOMETRIC_REPRESENTATION_ITEM()
RATIONAL_B_SPLINE_CURVE((1.7695059470837,1.7695059470837,1.66210638417258))
REPRESENTATION_ITEM('')
);
#4107=(
BOUNDED_CURVE()
B_SPLINE_CURVE(2,(#167430,#167431,#167432),.UNSPECIFIED.,.F.,.F.)
B_SPLINE_CURVE_WITH_KNOTS((3,3),(-1.90587960023829,-1.38751706971772),
 .UNSPECIFIED.)
CURVE()
GEOMETRIC_REPRESENTATION_ITEM()
RATIONAL_B_SPLINE_CURVE((1.66210638417239,1.7695059470837,1.7695059470837))
REPRESENTATION_ITEM('')
);
#4108=(
BOUNDED_CURVE()
B_SPLINE_CURVE(2,(#167444,#167445,#167446),.UNSPECIFIED.,.F.,.F.)
B_SPLINE_CURVE_WITH_KNOTS((3,3),(-1.38751706971772,-0.869154539197543),
 .UNSPECIFIED.)
CURVE()
GEOMETRIC_REPRESENTATION_ITEM()
RATIONAL_B_SPLINE_CURVE((1.7695059470837,1.7695059470837,1.66210638417255))
REPRESENTATION_ITEM('')
);
#4109=(
BOUNDED_CURVE()
B_SPLINE_CURVE(2,(#261646,#261647,#261648,#261649,#261650,#261651,#261652,
#261653,#261654,#261655,#261656,#261657,#261658,#261659,#261660),
 .UNSPECIFIED.,.F.,.F.)
B_SPLINE_CURVE_WITH_KNOTS((3,2,2,2,2,2,2,3),(0.75,0.7625,0.775,0.7875,0.8,
0.8125,0.825,0.832478990784214),.UNSPECIFIED.)
CURVE()
GEOMETRIC_REPRESENTATION_ITEM()
RATIONAL_B_SPLINE_CURVE((1.,0.923879532511287,1.,0.923879532511287,1.,0.923879532511287,
1.,0.923879532511287,1.,0.923879532511287,1.,0.923879532511287,1.,0.954455658012946,
0.963411430264977))
REPRESENTATION_ITEM('')
);
#4110=(
BOUNDED_CURVE()
B_SPLINE_CURVE(2,(#261663,#261664,#261665,#261666,#261667,#261668,#261669,
#261670,#261671,#261672,#261673,#261674,#261675,#261676,#261677),
 .UNSPECIFIED.,.F.,.F.)
B_SPLINE_CURVE_WITH_KNOTS((3,2,2,2,2,2,2,3),(0.75,0.7625,0.775,0.7875,0.8,
0.8125,0.825,0.832004152079254),.UNSPECIFIED.)
CURVE()
GEOMETRIC_REPRESENTATION_ITEM()
RATIONAL_B_SPLINE_CURVE((1.,0.923879532511287,1.,0.923879532511287,1.,0.923879532511287,
1.,0.923879532511287,1.,0.923879532511287,1.,0.923879532511287,1.,0.957347253549212,
0.962493918736692))
REPRESENTATION_ITEM('')
);
#4111=(
BOUNDED_CURVE()
B_SPLINE_CURVE(2,(#261682,#261683,#261684,#261685,#261686,#261687,#261688,
#261689,#261690,#261691,#261692,#261693,#261694,#261695,#261696,#261697,
#261698),.UNSPECIFIED.,.F.,.F.)
B_SPLINE_CURVE_WITH_KNOTS((3,2,2,2,2,2,2,2,3),(0.65,0.6625,0.675,0.6875,
0.7,0.7125,0.725,0.7375,0.75),.UNSPECIFIED.)
CURVE()
GEOMETRIC_REPRESENTATION_ITEM()
RATIONAL_B_SPLINE_CURVE((1.,0.923879532511287,1.,0.923879532511287,1.,0.923879532511287,
1.,0.923879532511287,1.,0.923879532511287,1.,0.923879532511287,1.,0.923879532511287,
1.,0.923879532511287,1.))
REPRESENTATION_ITEM('')
);
#4112=(
BOUNDED_CURVE()
B_SPLINE_CURVE(2,(#261699,#261700,#261701,#261702,#261703,#261704,#261705,
#261706,#261707,#261708,#261709,#261710,#261711,#261712,#261713,#261714,
#261715),.UNSPECIFIED.,.F.,.F.)
B_SPLINE_CURVE_WITH_KNOTS((3,2,2,2,2,2,2,2,3),(0.65,0.6625,0.675,0.6875,
0.7,0.7125,0.725,0.7375,0.75),.UNSPECIFIED.)
CURVE()
GEOMETRIC_REPRESENTATION_ITEM()
RATIONAL_B_SPLINE_CURVE((1.,0.923879532511287,1.,0.923879532511287,1.,0.923879532511287,
1.,0.923879532511287,1.,0.923879532511287,1.,0.923879532511287,1.,0.923879532511287,
1.,0.923879532511287,1.))
REPRESENTATION_ITEM('')
);
#4113=(
BOUNDED_CURVE()
B_SPLINE_CURVE(2,(#261720,#261721,#261722,#261723,#261724,#261725,#261726,
#261727,#261728,#261729,#261730,#261731,#261732,#261733,#261734,#261735,
#261736),.UNSPECIFIED.,.F.,.F.)
B_SPLINE_CURVE_WITH_KNOTS((3,2,2,2,2,2,2,2,3),(0.55,0.5625,0.575,0.5875,
0.6,0.6125,0.625,0.6375,0.65),.UNSPECIFIED.)
CURVE()
GEOMETRIC_REPRESENTATION_ITEM()
RATIONAL_B_SPLINE_CURVE((1.,0.923879532511287,1.,0.923879532511287,1.,0.923879532511287,
1.,0.923879532511287,1.,0.923879532511287,1.,0.923879532511287,1.,0.923879532511287,
1.,0.923879532511287,1.))
REPRESENTATION_ITEM('')
);
#4114=(
BOUNDED_CURVE()
B_SPLINE_CURVE(2,(#261737,#261738,#261739,#261740,#261741,#261742,#261743,
#261744,#261745,#261746,#261747,#261748,#261749,#261750,#261751,#261752,
#261753),.UNSPECIFIED.,.F.,.F.)
B_SPLINE_CURVE_WITH_KNOTS((3,2,2,2,2,2,2,2,3),(0.55,0.5625,0.575,0.5875,
0.6,0.6125,0.625,0.6375,0.65),.UNSPECIFIED.)
CURVE()
GEOMETRIC_REPRESENTATION_ITEM()
RATIONAL_B_SPLINE_CURVE((1.,0.923879532511287,1.,0.923879532511287,1.,0.923879532511287,
1.,0.923879532511287,1.,0.923879532511287,1.,0.923879532511287,1.,0.923879532511287,
1.,0.923879532511287,1.))
REPRESENTATION_ITEM('')
);
#4115=(
BOUNDED_CURVE()
B_SPLINE_CURVE(2,(#261758,#261759,#261760,#261761,#261762,#261763,#261764,
#261765,#261766,#261767,#261768,#261769,#261770,#261771,#261772,#261773,
#261774),.UNSPECIFIED.,.F.,.F.)
B_SPLINE_CURVE_WITH_KNOTS((3,2,2,2,2,2,2,2,3),(0.45,0.4625,0.475,0.4875,
0.5,0.5125,0.525,0.5375,0.55),.UNSPECIFIED.)
CURVE()
GEOMETRIC_REPRESENTATION_ITEM()
RATIONAL_B_SPLINE_CURVE((1.,0.923879532511287,1.,0.923879532511287,1.,0.923879532511287,
1.,0.923879532511287,1.,0.923879532511287,1.,0.923879532511287,1.,0.923879532511287,
1.,0.923879532511287,1.))
REPRESENTATION_ITEM('')
);
#4116=(
BOUNDED_CURVE()
B_SPLINE_CURVE(2,(#261775,#261776,#261777,#261778,#261779,#261780,#261781,
#261782,#261783,#261784,#261785,#261786,#261787,#261788,#261789,#261790,
#261791),.UNSPECIFIED.,.F.,.F.)
B_SPLINE_CURVE_WITH_KNOTS((3,2,2,2,2,2,2,2,3),(0.45,0.4625,0.475,0.4875,
0.5,0.5125,0.525,0.5375,0.55),.UNSPECIFIED.)
CURVE()
GEOMETRIC_REPRESENTATION_ITEM()
RATIONAL_B_SPLINE_CURVE((1.,0.923879532511287,1.,0.923879532511287,1.,0.923879532511287,
1.,0.923879532511287,1.,0.923879532511287,1.,0.923879532511287,1.,0.923879532511287,
1.,0.923879532511287,1.))
REPRESENTATION_ITEM('')
);
#4117=(
BOUNDED_CURVE()
B_SPLINE_CURVE(2,(#261796,#261797,#261798,#261799,#261800,#261801,#261802,
#261803,#261804,#261805,#261806,#261807,#261808,#261809,#261810,#261811,
#261812),.UNSPECIFIED.,.F.,.F.)
B_SPLINE_CURVE_WITH_KNOTS((3,2,2,2,2,2,2,2,3),(0.35,0.3625,0.375,0.3875,
0.4,0.4125,0.425,0.4375,0.45),.UNSPECIFIED.)
CURVE()
GEOMETRIC_REPRESENTATION_ITEM()
RATIONAL_B_SPLINE_CURVE((1.,0.923879532511287,1.,0.923879532511287,1.,0.923879532511287,
1.,0.923879532511287,1.,0.923879532511287,1.,0.923879532511287,1.,0.923879532511287,
1.,0.923879532511287,1.))
REPRESENTATION_ITEM('')
);
#4118=(
BOUNDED_CURVE()
B_SPLINE_CURVE(2,(#261813,#261814,#261815,#261816,#261817,#261818,#261819,
#261820,#261821,#261822,#261823,#261824,#261825,#261826,#261827,#261828,
#261829),.UNSPECIFIED.,.F.,.F.)
B_SPLINE_CURVE_WITH_KNOTS((3,2,2,2,2,2,2,2,3),(0.35,0.3625,0.375,0.3875,
0.4,0.4125,0.425,0.4375,0.45),.UNSPECIFIED.)
CURVE()
GEOMETRIC_REPRESENTATION_ITEM()
RATIONAL_B_SPLINE_CURVE((1.,0.923879532511287,1.,0.923879532511287,1.,0.923879532511287,
1.,0.923879532511287,1.,0.923879532511287,1.,0.923879532511287,1.,0.923879532511287,
1.,0.923879532511287,1.))
REPRESENTATION_ITEM('')
);
#4119=(
BOUNDED_CURVE()
B_SPLINE_CURVE(2,(#261834,#261835,#261836,#261837,#261838,#261839,#261840,
#261841,#261842,#261843,#261844,#261845,#261846,#261847,#261848,#261849,
#261850),.UNSPECIFIED.,.F.,.F.)
B_SPLINE_CURVE_WITH_KNOTS((3,2,2,2,2,2,2,2,3),(0.25,0.2625,0.275,0.2875,
0.3,0.3125,0.325,0.3375,0.35),.UNSPECIFIED.)
CURVE()
GEOMETRIC_REPRESENTATION_ITEM()
RATIONAL_B_SPLINE_CURVE((1.,0.923879532511287,1.,0.923879532511287,1.,0.923879532511287,
1.,0.923879532511287,1.,0.923879532511287,1.,0.923879532511287,1.,0.923879532511287,
1.,0.923879532511287,1.))
REPRESENTATION_ITEM('')
);
#4120=(
BOUNDED_CURVE()
B_SPLINE_CURVE(2,(#261851,#261852,#261853,#261854,#261855,#261856,#261857,
#261858,#261859,#261860,#261861,#261862,#261863,#261864,#261865,#261866,
#261867),.UNSPECIFIED.,.F.,.F.)
B_SPLINE_CURVE_WITH_KNOTS((3,2,2,2,2,2,2,2,3),(0.25,0.2625,0.275,0.2875,
0.3,0.3125,0.325,0.3375,0.35),.UNSPECIFIED.)
CURVE()
GEOMETRIC_REPRESENTATION_ITEM()
RATIONAL_B_SPLINE_CURVE((1.,0.923879532511287,1.,0.923879532511287,1.,0.923879532511287,
1.,0.923879532511287,1.,0.923879532511287,1.,0.923879532511287,1.,0.923879532511287,
1.,0.923879532511287,1.))
REPRESENTATION_ITEM('')
);
#4121=(
BOUNDED_CURVE()
B_SPLINE_CURVE(2,(#262441,#262442,#262443),.UNSPECIFIED.,.F.,.F.)
B_SPLINE_CURVE_WITH_KNOTS((3,3),(-0.50202782853392,-0.138654436681084),
 .UNSPECIFIED.)
CURVE()
GEOMETRIC_REPRESENTATION_ITEM()
RATIONAL_B_SPLINE_CURVE((1.19489831606823,1.37974972887269,1.19489831606823))
REPRESENTATION_ITEM('')
);
#4122=(
BOUNDED_CURVE()
B_SPLINE_CURVE(2,(#262445,#262446,#262447),.UNSPECIFIED.,.F.,.F.)
B_SPLINE_CURVE_WITH_KNOTS((3,3),(-0.502027828533919,-0.138654436681081),
 .UNSPECIFIED.)
CURVE()
GEOMETRIC_REPRESENTATION_ITEM()
RATIONAL_B_SPLINE_CURVE((1.19489831606823,1.3797497288727,1.19489831606823))
REPRESENTATION_ITEM('')
);
#4123=(
BOUNDED_CURVE()
B_SPLINE_CURVE(2,(#262449,#262450,#262451),.UNSPECIFIED.,.F.,.F.)
B_SPLINE_CURVE_WITH_KNOTS((3,3),(-0.502027828533919,-0.138654436681082),
 .UNSPECIFIED.)
CURVE()
GEOMETRIC_REPRESENTATION_ITEM()
RATIONAL_B_SPLINE_CURVE((1.19489831606824,1.37974972887271,1.19489831606824))
REPRESENTATION_ITEM('')
);
#4124=(
BOUNDED_CURVE()
B_SPLINE_CURVE(2,(#262453,#262454,#262455),.UNSPECIFIED.,.F.,.F.)
B_SPLINE_CURVE_WITH_KNOTS((3,3),(-0.502027828533919,-0.138654436681086),
 .UNSPECIFIED.)
CURVE()
GEOMETRIC_REPRESENTATION_ITEM()
RATIONAL_B_SPLINE_CURVE((1.19489831606823,1.37974972887268,1.19489831606823))
REPRESENTATION_ITEM('')
);
#4125=(
BOUNDED_CURVE()
B_SPLINE_CURVE(2,(#262457,#262458,#262459),.UNSPECIFIED.,.F.,.F.)
B_SPLINE_CURVE_WITH_KNOTS((3,3),(-0.502027828533918,-0.138654436681083),
 .UNSPECIFIED.)
CURVE()
GEOMETRIC_REPRESENTATION_ITEM()
RATIONAL_B_SPLINE_CURVE((1.19489831606823,1.3797497288727,1.19489831606823))
REPRESENTATION_ITEM('')
);
#4126=(
BOUNDED_CURVE()
B_SPLINE_CURVE(2,(#262461,#262462,#262463),.UNSPECIFIED.,.F.,.F.)
B_SPLINE_CURVE_WITH_KNOTS((3,3),(-0.502027828533914,-0.138654436681084),
 .UNSPECIFIED.)
CURVE()
GEOMETRIC_REPRESENTATION_ITEM()
RATIONAL_B_SPLINE_CURVE((1.19489831606823,1.37974972887268,1.19489831606822))
REPRESENTATION_ITEM('')
);
#4127=(
BOUNDED_CURVE()
B_SPLINE_CURVE(2,(#262811,#262812,#262813,#262814,#262815,#262816,#262817,
#262818,#262819,#262820,#262821,#262822,#262823,#262824,#262825,#262826,
#262827),.UNSPECIFIED.,.F.,.F.)
B_SPLINE_CURVE_WITH_KNOTS((3,2,2,2,2,2,2,2,3),(0.152008120250914,0.1625,
0.175,0.1875,0.2,0.2125,0.225,0.2375,0.25),.UNSPECIFIED.)
CURVE()
GEOMETRIC_REPRESENTATION_ITEM()
RATIONAL_B_SPLINE_CURVE((0.979471631423889,0.936108256693134,1.,0.923879532511287,
1.,0.923879532511287,1.,0.923879532511287,1.,0.923879532511287,1.,0.923879532511287,
1.,0.923879532511287,1.,0.923879532511287,1.))
REPRESENTATION_ITEM('')
);
#4128=(
BOUNDED_CURVE()
B_SPLINE_CURVE(2,(#262829,#262830,#262831,#262832,#262833,#262834,#262835,
#262836,#262837,#262838,#262839,#262840,#262841,#262842,#262843,#262844,
#262845),.UNSPECIFIED.,.F.,.F.)
B_SPLINE_CURVE_WITH_KNOTS((3,2,2,2,2,2,2,2,3),(0.152504986222125,0.1625,
0.175,0.1875,0.2,0.2125,0.225,0.2375,0.25),.UNSPECIFIED.)
CURVE()
GEOMETRIC_REPRESENTATION_ITEM()
RATIONAL_B_SPLINE_CURVE((0.975605037486425,0.939133990293761,1.,0.923879532511287,
1.,0.923879532511287,1.,0.923879532511287,1.,0.923879532511287,1.,0.923879532511287,
1.,0.923879532511287,1.,0.923879532511287,1.))
REPRESENTATION_ITEM('')
);
#4129=(
BOUNDED_CURVE()
B_SPLINE_CURVE(2,(#263173,#263174,#263175,#263176,#263177,#263178,#263179,
#263180,#263181,#263182,#263183,#263184,#263185,#263186,#263187),
 .UNSPECIFIED.,.F.,.F.)
B_SPLINE_CURVE_WITH_KNOTS((3,2,2,2,2,2,2,3),(0.75,0.7625,0.775,0.7875,0.8,
0.8125,0.825,0.832478990784214),.UNSPECIFIED.)
CURVE()
GEOMETRIC_REPRESENTATION_ITEM()
RATIONAL_B_SPLINE_CURVE((1.,0.923879532511287,1.,0.923879532511287,1.,0.923879532511287,
1.,0.923879532511287,1.,0.923879532511287,1.,0.923879532511287,1.,0.954455658012946,
0.963411430264977))
REPRESENTATION_ITEM('')
);
#4130=(
BOUNDED_CURVE()
B_SPLINE_CURVE(2,(#263190,#263191,#263192,#263193,#263194,#263195,#263196,
#263197,#263198,#263199,#263200,#263201,#263202,#263203,#263204),
 .UNSPECIFIED.,.F.,.F.)
B_SPLINE_CURVE_WITH_KNOTS((3,2,2,2,2,2,2,3),(0.75,0.7625,0.775,0.7875,0.8,
0.8125,0.825,0.832004152079254),.UNSPECIFIED.)
CURVE()
GEOMETRIC_REPRESENTATION_ITEM()
RATIONAL_B_SPLINE_CURVE((1.,0.923879532511287,1.,0.923879532511287,1.,0.923879532511287,
1.,0.923879532511287,1.,0.923879532511287,1.,0.923879532511287,1.,0.957347253549212,
0.962493918736692))
REPRESENTATION_ITEM('')
);
#4131=(
BOUNDED_CURVE()
B_SPLINE_CURVE(2,(#263209,#263210,#263211,#263212,#263213,#263214,#263215,
#263216,#263217,#263218,#263219,#263220,#263221,#263222,#263223,#263224,
#263225),.UNSPECIFIED.,.F.,.F.)
B_SPLINE_CURVE_WITH_KNOTS((3,2,2,2,2,2,2,2,3),(0.65,0.6625,0.675,0.6875,
0.7,0.7125,0.725,0.7375,0.75),.UNSPECIFIED.)
CURVE()
GEOMETRIC_REPRESENTATION_ITEM()
RATIONAL_B_SPLINE_CURVE((1.,0.923879532511287,1.,0.923879532511287,1.,0.923879532511287,
1.,0.923879532511287,1.,0.923879532511287,1.,0.923879532511287,1.,0.923879532511287,
1.,0.923879532511287,1.))
REPRESENTATION_ITEM('')
);
#4132=(
BOUNDED_CURVE()
B_SPLINE_CURVE(2,(#263226,#263227,#263228,#263229,#263230,#263231,#263232,
#263233,#263234,#263235,#263236,#263237,#263238,#263239,#263240,#263241,
#263242),.UNSPECIFIED.,.F.,.F.)
B_SPLINE_CURVE_WITH_KNOTS((3,2,2,2,2,2,2,2,3),(0.65,0.6625,0.675,0.6875,
0.7,0.7125,0.725,0.7375,0.75),.UNSPECIFIED.)
CURVE()
GEOMETRIC_REPRESENTATION_ITEM()
RATIONAL_B_SPLINE_CURVE((1.,0.923879532511287,1.,0.923879532511287,1.,0.923879532511287,
1.,0.923879532511287,1.,0.923879532511287,1.,0.923879532511287,1.,0.923879532511287,
1.,0.923879532511287,1.))
REPRESENTATION_ITEM('')
);
#4133=(
BOUNDED_CURVE()
B_SPLINE_CURVE(2,(#263247,#263248,#263249,#263250,#263251,#263252,#263253,
#263254,#263255,#263256,#263257,#263258,#263259,#263260,#263261,#263262,
#263263),.UNSPECIFIED.,.F.,.F.)
B_SPLINE_CURVE_WITH_KNOTS((3,2,2,2,2,2,2,2,3),(0.55,0.5625,0.575,0.5875,
0.6,0.6125,0.625,0.6375,0.65),.UNSPECIFIED.)
CURVE()
GEOMETRIC_REPRESENTATION_ITEM()
RATIONAL_B_SPLINE_CURVE((1.,0.923879532511287,1.,0.923879532511287,1.,0.923879532511287,
1.,0.923879532511287,1.,0.923879532511287,1.,0.923879532511287,1.,0.923879532511287,
1.,0.923879532511287,1.))
REPRESENTATION_ITEM('')
);
#4134=(
BOUNDED_CURVE()
B_SPLINE_CURVE(2,(#263264,#263265,#263266,#263267,#263268,#263269,#263270,
#263271,#263272,#263273,#263274,#263275,#263276,#263277,#263278,#263279,
#263280),.UNSPECIFIED.,.F.,.F.)
B_SPLINE_CURVE_WITH_KNOTS((3,2,2,2,2,2,2,2,3),(0.55,0.5625,0.575,0.5875,
0.6,0.6125,0.625,0.6375,0.65),.UNSPECIFIED.)
CURVE()
GEOMETRIC_REPRESENTATION_ITEM()
RATIONAL_B_SPLINE_CURVE((1.,0.923879532511287,1.,0.923879532511287,1.,0.923879532511287,
1.,0.923879532511287,1.,0.923879532511287,1.,0.923879532511287,1.,0.923879532511287,
1.,0.923879532511287,1.))
REPRESENTATION_ITEM('')
);
#4135=(
BOUNDED_CURVE()
B_SPLINE_CURVE(2,(#263285,#263286,#263287,#263288,#263289,#263290,#263291,
#263292,#263293,#263294,#263295,#263296,#263297,#263298,#263299,#263300,
#263301),.UNSPECIFIED.,.F.,.F.)
B_SPLINE_CURVE_WITH_KNOTS((3,2,2,2,2,2,2,2,3),(0.45,0.4625,0.475,0.4875,
0.5,0.5125,0.525,0.5375,0.55),.UNSPECIFIED.)
CURVE()
GEOMETRIC_REPRESENTATION_ITEM()
RATIONAL_B_SPLINE_CURVE((1.,0.923879532511287,1.,0.923879532511287,1.,0.923879532511287,
1.,0.923879532511287,1.,0.923879532511287,1.,0.923879532511287,1.,0.923879532511287,
1.,0.923879532511287,1.))
REPRESENTATION_ITEM('')
);
#4136=(
BOUNDED_CURVE()
B_SPLINE_CURVE(2,(#263302,#263303,#263304,#263305,#263306,#263307,#263308,
#263309,#263310,#263311,#263312,#263313,#263314,#263315,#263316,#263317,
#263318),.UNSPECIFIED.,.F.,.F.)
B_SPLINE_CURVE_WITH_KNOTS((3,2,2,2,2,2,2,2,3),(0.45,0.4625,0.475,0.4875,
0.5,0.5125,0.525,0.5375,0.55),.UNSPECIFIED.)
CURVE()
GEOMETRIC_REPRESENTATION_ITEM()
RATIONAL_B_SPLINE_CURVE((1.,0.923879532511287,1.,0.923879532511287,1.,0.923879532511287,
1.,0.923879532511287,1.,0.923879532511287,1.,0.923879532511287,1.,0.923879532511287,
1.,0.923879532511287,1.))
REPRESENTATION_ITEM('')
);
#4137=(
BOUNDED_CURVE()
B_SPLINE_CURVE(2,(#263323,#263324,#263325,#263326,#263327,#263328,#263329,
#263330,#263331,#263332,#263333,#263334,#263335,#263336,#263337,#263338,
#263339),.UNSPECIFIED.,.F.,.F.)
B_SPLINE_CURVE_WITH_KNOTS((3,2,2,2,2,2,2,2,3),(0.35,0.3625,0.375,0.3875,
0.4,0.4125,0.425,0.4375,0.45),.UNSPECIFIED.)
CURVE()
GEOMETRIC_REPRESENTATION_ITEM()
RATIONAL_B_SPLINE_CURVE((1.,0.923879532511287,1.,0.923879532511287,1.,0.923879532511287,
1.,0.923879532511287,1.,0.923879532511287,1.,0.923879532511287,1.,0.923879532511287,
1.,0.923879532511287,1.))
REPRESENTATION_ITEM('')
);
#4138=(
BOUNDED_CURVE()
B_SPLINE_CURVE(2,(#263340,#263341,#263342,#263343,#263344,#263345,#263346,
#263347,#263348,#263349,#263350,#263351,#263352,#263353,#263354,#263355,
#263356),.UNSPECIFIED.,.F.,.F.)
B_SPLINE_CURVE_WITH_KNOTS((3,2,2,2,2,2,2,2,3),(0.35,0.3625,0.375,0.3875,
0.4,0.4125,0.425,0.4375,0.45),.UNSPECIFIED.)
CURVE()
GEOMETRIC_REPRESENTATION_ITEM()
RATIONAL_B_SPLINE_CURVE((1.,0.923879532511287,1.,0.923879532511287,1.,0.923879532511287,
1.,0.923879532511287,1.,0.923879532511287,1.,0.923879532511287,1.,0.923879532511287,
1.,0.923879532511287,1.))
REPRESENTATION_ITEM('')
);
#4139=(
BOUNDED_CURVE()
B_SPLINE_CURVE(2,(#263361,#263362,#263363,#263364,#263365,#263366,#263367,
#263368,#263369,#263370,#263371,#263372,#263373,#263374,#263375,#263376,
#263377),.UNSPECIFIED.,.F.,.F.)
B_SPLINE_CURVE_WITH_KNOTS((3,2,2,2,2,2,2,2,3),(0.25,0.2625,0.275,0.2875,
0.3,0.3125,0.325,0.3375,0.35),.UNSPECIFIED.)
CURVE()
GEOMETRIC_REPRESENTATION_ITEM()
RATIONAL_B_SPLINE_CURVE((1.,0.923879532511287,1.,0.923879532511287,1.,0.923879532511287,
1.,0.923879532511287,1.,0.923879532511287,1.,0.923879532511287,1.,0.923879532511287,
1.,0.923879532511287,1.))
REPRESENTATION_ITEM('')
);
#4140=(
BOUNDED_CURVE()
B_SPLINE_CURVE(2,(#263378,#263379,#263380,#263381,#263382,#263383,#263384,
#263385,#263386,#263387,#263388,#263389,#263390,#263391,#263392,#263393,
#263394),.UNSPECIFIED.,.F.,.F.)
B_SPLINE_CURVE_WITH_KNOTS((3,2,2,2,2,2,2,2,3),(0.25,0.2625,0.275,0.2875,
0.3,0.3125,0.325,0.3375,0.35),.UNSPECIFIED.)
CURVE()
GEOMETRIC_REPRESENTATION_ITEM()
RATIONAL_B_SPLINE_CURVE((1.,0.923879532511287,1.,0.923879532511287,1.,0.923879532511287,
1.,0.923879532511287,1.,0.923879532511287,1.,0.923879532511287,1.,0.923879532511287,
1.,0.923879532511287,1.))
REPRESENTATION_ITEM('')
);
#4141=(
BOUNDED_CURVE()
B_SPLINE_CURVE(2,(#263968,#263969,#263970),.UNSPECIFIED.,.F.,.F.)
B_SPLINE_CURVE_WITH_KNOTS((3,3),(-0.502027828533916,-0.138654436681082),
 .UNSPECIFIED.)
CURVE()
GEOMETRIC_REPRESENTATION_ITEM()
RATIONAL_B_SPLINE_CURVE((1.19489831606823,1.3797497288727,1.19489831606823))
REPRESENTATION_ITEM('')
);
#4142=(
BOUNDED_CURVE()
B_SPLINE_CURVE(2,(#263972,#263973,#263974),.UNSPECIFIED.,.F.,.F.)
B_SPLINE_CURVE_WITH_KNOTS((3,3),(-0.50202782853392,-0.138654436681083),
 .UNSPECIFIED.)
CURVE()
GEOMETRIC_REPRESENTATION_ITEM()
RATIONAL_B_SPLINE_CURVE((1.19489831606823,1.3797497288727,1.19489831606823))
REPRESENTATION_ITEM('')
);
#4143=(
BOUNDED_CURVE()
B_SPLINE_CURVE(2,(#263976,#263977,#263978),.UNSPECIFIED.,.F.,.F.)
B_SPLINE_CURVE_WITH_KNOTS((3,3),(-0.502027828533917,-0.138654436681082),
 .UNSPECIFIED.)
CURVE()
GEOMETRIC_REPRESENTATION_ITEM()
RATIONAL_B_SPLINE_CURVE((1.19489831606823,1.3797497288727,1.19489831606823))
REPRESENTATION_ITEM('')
);
#4144=(
BOUNDED_CURVE()
B_SPLINE_CURVE(2,(#263980,#263981,#263982),.UNSPECIFIED.,.F.,.F.)
B_SPLINE_CURVE_WITH_KNOTS((3,3),(-0.502027828533925,-0.138654436681083),
 .UNSPECIFIED.)
CURVE()
GEOMETRIC_REPRESENTATION_ITEM()
RATIONAL_B_SPLINE_CURVE((1.19489831606823,1.37974972887271,1.19489831606823))
REPRESENTATION_ITEM('')
);
#4145=(
BOUNDED_CURVE()
B_SPLINE_CURVE(2,(#263984,#263985,#263986),.UNSPECIFIED.,.F.,.F.)
B_SPLINE_CURVE_WITH_KNOTS((3,3),(-0.502027828533916,-0.138654436681082),
 .UNSPECIFIED.)
CURVE()
GEOMETRIC_REPRESENTATION_ITEM()
RATIONAL_B_SPLINE_CURVE((1.19489831606823,1.3797497288727,1.19489831606823))
REPRESENTATION_ITEM('')
);
#4146=(
BOUNDED_CURVE()
B_SPLINE_CURVE(2,(#263988,#263989,#263990),.UNSPECIFIED.,.F.,.F.)
B_SPLINE_CURVE_WITH_KNOTS((3,3),(-0.502027828533915,-0.138654436681083),
 .UNSPECIFIED.)
CURVE()
GEOMETRIC_REPRESENTATION_ITEM()
RATIONAL_B_SPLINE_CURVE((1.19489831606823,1.3797497288727,1.19489831606823))
REPRESENTATION_ITEM('')
);
#4147=(
BOUNDED_CURVE()
B_SPLINE_CURVE(2,(#264338,#264339,#264340,#264341,#264342,#264343,#264344,
#264345,#264346,#264347,#264348,#264349,#264350,#264351,#264352,#264353,
#264354),.UNSPECIFIED.,.F.,.F.)
B_SPLINE_CURVE_WITH_KNOTS((3,2,2,2,2,2,2,2,3),(0.152008120250914,0.1625,
0.175,0.1875,0.2,0.2125,0.225,0.2375,0.25),.UNSPECIFIED.)
CURVE()
GEOMETRIC_REPRESENTATION_ITEM()
RATIONAL_B_SPLINE_CURVE((0.979471631423889,0.936108256693134,1.,0.923879532511287,
1.,0.923879532511287,1.,0.923879532511287,1.,0.923879532511287,1.,0.923879532511287,
1.,0.923879532511287,1.,0.923879532511287,1.))
REPRESENTATION_ITEM('')
);
#4148=(
BOUNDED_CURVE()
B_SPLINE_CURVE(2,(#264356,#264357,#264358,#264359,#264360,#264361,#264362,
#264363,#264364,#264365,#264366,#264367,#264368,#264369,#264370,#264371,
#264372),.UNSPECIFIED.,.F.,.F.)
B_SPLINE_CURVE_WITH_KNOTS((3,2,2,2,2,2,2,2,3),(0.152504986222125,0.1625,
0.175,0.1875,0.2,0.2125,0.225,0.2375,0.25),.UNSPECIFIED.)
CURVE()
GEOMETRIC_REPRESENTATION_ITEM()
RATIONAL_B_SPLINE_CURVE((0.975605037486425,0.939133990293761,1.,0.923879532511287,
1.,0.923879532511287,1.,0.923879532511287,1.,0.923879532511287,1.,0.923879532511287,
1.,0.923879532511287,1.,0.923879532511287,1.))
REPRESENTATION_ITEM('')
);
#4243=B_SPLINE_CURVE_WITH_KNOTS('',3,(#167156,#167157,#167158,#167159,#167160,
#167161,#167162,#167163,#167164,#167165),.UNSPECIFIED.,.F.,.F.,(4,2,2,2,
4),(0.06129084465535,0.0663539220633962,0.0872647966493331,0.10817567123527,
0.113238748643028),.UNSPECIFIED.);
#4244=B_SPLINE_CURVE_WITH_KNOTS('',3,(#167169,#167170,#167171,#167172,#167173,
#167174,#167175,#167176,#167177,#167178),.UNSPECIFIED.,.F.,.F.,(4,2,2,2,
4),(0.21714824555634,0.222211322964386,0.243122197550323,0.26403307213626,
0.269096149544019),.UNSPECIFIED.);
#4245=B_SPLINE_CURVE_WITH_KNOTS('',3,(#167205,#167206,#167207,#167208,#167209,
#167210,#167211,#167212,#167213,#167214),.UNSPECIFIED.,.F.,.F.,(4,2,2,2,
4),(-0.113238748643028,-0.10817567123527,-0.0872647966493331,-0.0663539220633962,
-0.0612908446553502),.UNSPECIFIED.);
#4246=B_SPLINE_CURVE_WITH_KNOTS('',3,(#167271,#167272,#167273,#167274,#167275,
#167276,#167277,#167278,#167279,#167280),.UNSPECIFIED.,.F.,.F.,(4,2,2,2,
4),(-0.113238748643275,-0.10817567123527,-0.0872647966493331,-0.0663539220633962,
-0.061290844655351),.UNSPECIFIED.);
#4247=B_SPLINE_CURVE_WITH_KNOTS('',3,(#167290,#167291,#167292,#167293,#167294,
#167295,#167296,#167297,#167298,#167299),.UNSPECIFIED.,.F.,.F.,(4,2,2,2,
4),(-0.113238748643028,-0.10817567123527,-0.0872647966493333,-0.0663539220633963,
-0.061290844655349),.UNSPECIFIED.);
#4248=B_SPLINE_CURVE_WITH_KNOTS('',3,(#167309,#167310,#167311,#167312,#167313,
#167314,#167315,#167316,#167317,#167318),.UNSPECIFIED.,.F.,.F.,(4,2,2,2,
4),(-0.113238748643316,-0.10817567123527,-0.0872647966493333,-0.0663539220633963,
-0.0612908446553511),.UNSPECIFIED.);
#4249=B_SPLINE_CURVE_WITH_KNOTS('',3,(#167328,#167329,#167330,#167331,#167332,
#167333,#167334,#167335,#167336,#167337),.UNSPECIFIED.,.F.,.F.,(4,2,2,2,
4),(-0.113238748643028,-0.10817567123527,-0.0872647966493333,-0.0663539220633963,
-0.0612908446553899),.UNSPECIFIED.);
#4250=B_SPLINE_CURVE_WITH_KNOTS('',3,(#167358,#167359,#167360,#167361,#167362,
#167363,#167364,#167365,#167366,#167367),.UNSPECIFIED.,.F.,.F.,(4,2,2,2,
4),(-0.269096149544267,-0.26403307213626,-0.243122197550323,-0.222211322964386,
-0.21714824555634),.UNSPECIFIED.);
#4251=B_SPLINE_CURVE_WITH_KNOTS('',3,(#167377,#167378,#167379,#167380,#167381,
#167382,#167383,#167384,#167385,#167386),.UNSPECIFIED.,.F.,.F.,(4,2,2,2,
4),(-0.269096149544016,-0.26403307213626,-0.243122197550323,-0.222211322964386,
-0.217148245556339),.UNSPECIFIED.);
#4252=B_SPLINE_CURVE_WITH_KNOTS('',3,(#167396,#167397,#167398,#167399,#167400,
#167401,#167402,#167403,#167404,#167405),.UNSPECIFIED.,.F.,.F.,(4,2,2,2,
4),(-0.269096149544018,-0.26403307213626,-0.243122197550323,-0.222211322964386,
-0.21714824555634),.UNSPECIFIED.);
#4253=B_SPLINE_CURVE_WITH_KNOTS('',3,(#167415,#167416,#167417,#167418,#167419,
#167420,#167421,#167422,#167423,#167424),.UNSPECIFIED.,.F.,.F.,(4,2,2,2,
4),(-0.269096149544306,-0.26403307213626,-0.243122197550323,-0.222211322964386,
-0.21714824555634),.UNSPECIFIED.);
#4254=B_SPLINE_CURVE_WITH_KNOTS('',3,(#167434,#167435,#167436,#167437,#167438,
#167439,#167440,#167441,#167442,#167443),.UNSPECIFIED.,.F.,.F.,(4,2,2,2,
4),(-0.269096149544019,-0.26403307213626,-0.243122197550323,-0.222211322964386,
-0.217148245556379),.UNSPECIFIED.);
#4255=B_SPLINE_CURVE_WITH_KNOTS('',3,(#167669,#167670,#167671,#167672,#167673,
#167674,#167675,#167676,#167677,#167678,#167679,#167680,#167681,#167682,
#167683,#167684,#167685,#167686,#167687,#167688,#167689,#167690,#167691,
#167692,#167693,#167694,#167695,#167696,#167697,#167698,#167699,#167700,
#167701,#167702,#167703,#167704,#167705,#167706,#167707,#167708,#167709,
#167710,#167711),.UNSPECIFIED.,.F.,.F.,(4,3,3,3,3,3,3,3,3,3,3,3,3,3,4),
(1.00966327312713E-18,1.12890698065757E-5,7.65259667098946E-5,0.000102837507928451,
0.000112544869199196,0.000130746171581843,0.000194450729921106,0.000226303009090737,
0.000242229148675553,0.000258155288260369,0.000258291104876507,0.00032765463360993,
0.000399363990826254,0.00046970928517733,0.000516310576520721),
 .UNSPECIFIED.);
#4256=B_SPLINE_CURVE_WITH_KNOTS('',3,(#167719,#167720,#167721,#167722,#167723,
#167724,#167725,#167726,#167727,#167728,#167729,#167730,#167731,#167732,
#167733,#167734,#167735,#167736,#167737,#167738,#167739,#167740,#167741,
#167742,#167743,#167744,#167745,#167746,#167747,#167748,#167749,#167750,
#167751,#167752,#167753,#167754,#167755,#167756,#167757,#167758),
 .UNSPECIFIED.,.F.,.F.,(4,3,3,3,3,3,3,3,3,3,3,3,3,4),(1.20009527741861E-17,
6.84564250799994E-5,0.000138288406590926,0.000205407478924308,0.000256966021225851,
0.000257101146970264,0.000271589374668168,0.00035221306761286,0.000388398097499794,
0.000404123622054885,0.000459162957997706,0.000486682625969117,0.000500442459954822,
0.000514202293940527),.UNSPECIFIED.);
#4257=B_SPLINE_CURVE_WITH_KNOTS('',3,(#167762,#167763,#167764,#167765,#167766,
#167767,#167768,#167769,#167770,#167771,#167772,#167773,#167774,#167775,
#167776,#167777,#167778,#167779,#167780,#167781,#167782,#167783,#167784,
#167785,#167786,#167787,#167788,#167789,#167790,#167791,#167792,#167793,
#167794,#167795,#167796,#167797,#167798,#167799,#167800,#167801,#167802,
#167803,#167804),.UNSPECIFIED.,.F.,.F.,(4,3,3,3,3,3,3,3,3,3,3,3,3,3,4),
(8.67361737988403E-19,1.12890698065828E-5,7.65259666997707E-5,0.000102837507928519,
0.00011254486919926,0.000130746171581899,0.000194450729921135,0.000226303009090753,
0.000242229148675562,0.000258155288260372,0.000258291104876513,0.000327654633625812,
0.000399363990857997,0.000469709285222688,0.000516310576520742),
 .UNSPECIFIED.);
#4258=B_SPLINE_CURVE_WITH_KNOTS('',3,(#167812,#167813,#167814,#167815,#167816,
#167817,#167818,#167819,#167820,#167821,#167822,#167823,#167824,#167825,
#167826,#167827,#167828,#167829,#167830,#167831,#167832,#167833,#167834,
#167835,#167836,#167837,#167838,#167839,#167840,#167841,#167842,#167843,
#167844,#167845,#167846,#167847,#167848,#167849,#167850,#167851),
 .UNSPECIFIED.,.F.,.F.,(4,3,3,3,3,3,3,3,3,3,3,3,3,4),(0.,6.84564250830358E-5,
0.00013828840659705,0.000205407478933295,0.000256966021225846,0.000257101146970262,
0.000271589374668165,0.000352213067609841,0.000388398097499827,0.000404123622054914,
0.000459162957997719,0.000486682625969121,0.000500442459954823,0.000514202293940524),
 .UNSPECIFIED.);
#4259=B_SPLINE_CURVE_WITH_KNOTS('',3,(#167855,#167856,#167857,#167858,#167859,
#167860,#167861,#167862,#167863,#167864,#167865,#167866,#167867,#167868,
#167869,#167870,#167871,#167872,#167873,#167874,#167875,#167876,#167877,
#167878,#167879,#167880,#167881,#167882,#167883,#167884,#167885,#167886,
#167887,#167888,#167889,#167890,#167891,#167892,#167893,#167894,#167895,
#167896,#167897),.UNSPECIFIED.,.F.,.F.,(4,3,3,3,3,3,3,3,3,3,3,3,3,3,4),
(1.73472347597681E-18,1.12890698065783E-5,7.65259667045031E-5,0.000102837507928451,
0.000112544869199196,0.000130746171581843,0.000194450729921108,0.00022630300909074,
0.000242229148675556,0.000258155288260373,0.000258291104876516,0.000327654633619643,
0.000399363990846141,0.000469709285206287,0.000516310576520743),
 .UNSPECIFIED.);
#4260=B_SPLINE_CURVE_WITH_KNOTS('',3,(#167905,#167906,#167907,#167908,#167909,
#167910,#167911,#167912,#167913,#167914,#167915,#167916,#167917,#167918,
#167919,#167920,#167921,#167922,#167923,#167924,#167925,#167926,#167927,
#167928,#167929,#167930,#167931,#167932,#167933,#167934,#167935,#167936,
#167937,#167938,#167939,#167940,#167941,#167942,#167943,#167944),
 .UNSPECIFIED.,.F.,.F.,(4,3,3,3,3,3,3,3,3,3,3,3,3,4),(0.,6.84564250848561E-5,
0.000138288406600877,0.00020540747893902,0.000256966021225847,0.00025710114697026,
0.00027158937466817,0.000352213067607056,0.000388398097499874,0.000404123622054955,
0.000459162957997738,0.000486682625969129,0.000500442459954825,0.000514202293940521),
 .UNSPECIFIED.);
#4261=B_SPLINE_CURVE_WITH_KNOTS('',3,(#167948,#167949,#167950,#167951,#167952,
#167953,#167954,#167955,#167956,#167957,#167958,#167959,#167960,#167961,
#167962,#167963,#167964,#167965,#167966,#167967,#167968,#167969,#167970,
#167971,#167972,#167973,#167974,#167975,#167976,#167977,#167978,#167979,
#167980,#167981,#167982,#167983,#167984,#167985,#167986,#167987,#167988,
#167989,#167990),.UNSPECIFIED.,.F.,.F.,(4,3,3,3,3,3,3,3,3,3,3,3,3,3,4),
(0.,1.12890698065866E-5,7.65259667154617E-5,0.000102837507928558,0.000112544869199297,
0.000130746171581931,0.000194450729921151,0.000226303009090762,0.000242229148675567,
0.000258155288260372,0.000258291104876507,0.000327654633617086,0.000399363990840721,
0.000469709285197883,0.000516310576520743),.UNSPECIFIED.);
#4262=B_SPLINE_CURVE_WITH_KNOTS('',3,(#167998,#167999,#168000,#168001,#168002,
#168003,#168004,#168005,#168006,#168007,#168008,#168009,#168010,#168011,
#168012,#168013,#168014,#168015,#168016,#168017,#168018,#168019,#168020,
#168021,#168022,#168023,#168024,#168025,#168026,#168027,#168028,#168029,
#168030,#168031,#168032,#168033,#168034,#168035,#168036,#168037),
 .UNSPECIFIED.,.F.,.F.,(4,3,3,3,3,3,3,3,3,3,3,3,3,4),(0.,6.84564250816342E-5,
0.000138288406594322,0.000205407478929741,0.000256966021225855,0.000257101146970265,
0.000271589374668173,0.000352213067599976,0.000388398097499811,0.0004041236220549,
0.000459162957997715,0.000486682625969123,0.000500442459954826,0.00051420229394053),
 .UNSPECIFIED.);
#4263=B_SPLINE_CURVE_WITH_KNOTS('',3,(#168041,#168042,#168043,#168044,#168045,
#168046,#168047,#168048,#168049,#168050,#168051,#168052,#168053,#168054,
#168055,#168056,#168057,#168058,#168059,#168060,#168061,#168062,#168063,
#168064,#168065,#168066,#168067,#168068,#168069,#168070,#168071,#168072,
#168073,#168074,#168075,#168076,#168077,#168078,#168079,#168080,#168081,
#168082,#168083),.UNSPECIFIED.,.F.,.F.,(4,3,3,3,3,3,3,3,3,3,3,3,3,3,4),
(3.46944695195361E-18,1.12890698065793E-5,7.65259667061472E-5,0.000102837507928427,
0.000112544869199174,0.000130746171581824,0.000194450729921099,0.000226303009090737,
0.000242229148675555,0.000258155288260374,0.000258291104876507,0.000327654633615792,
0.000399363990838126,0.000469709285194437,0.000516310576520745),
 .UNSPECIFIED.);
#4264=B_SPLINE_CURVE_WITH_KNOTS('',3,(#168091,#168092,#168093,#168094,#168095,
#168096,#168097,#168098,#168099,#168100,#168101,#168102,#168103,#168104,
#168105,#168106,#168107,#168108,#168109,#168110,#168111,#168112,#168113,
#168114,#168115,#168116,#168117,#168118,#168119,#168120,#168121,#168122,
#168123,#168124,#168125,#168126,#168127,#168128,#168129,#168130),
 .UNSPECIFIED.,.F.,.F.,(4,3,3,3,3,3,3,3,3,3,3,3,3,4),(0.,6.84564250791255E-5,
0.000138288406588817,0.000205407478920826,0.000256966021225839,0.000257101146970257,
0.000271589374668167,0.000352213067604686,0.00038839809749988,0.00040412362205496,
0.000459162957997741,0.000486682625969131,0.000500442459954827,0.000514202293940522),
 .UNSPECIFIED.);
#4265=B_SPLINE_CURVE_WITH_KNOTS('',3,(#168134,#168135,#168136,#168137,#168138,
#168139,#168140,#168141,#168142,#168143,#168144,#168145,#168146,#168147,
#168148,#168149,#168150,#168151,#168152,#168153,#168154,#168155,#168156,
#168157,#168158,#168159,#168160,#168161,#168162,#168163,#168164,#168165,
#168166,#168167,#168168,#168169,#168170,#168171,#168172,#168173,#168174,
#168175,#168176),.UNSPECIFIED.,.F.,.F.,(4,3,3,3,3,3,3,3,3,3,3,3,3,3,4),
(0.,1.128906980658E-5,7.65259667055946E-5,0.000102837507928488,0.000112544869199231,
0.000130746171581874,0.000194450729921126,0.000226303009090752,0.000242229148675565,
0.000258155288260378,0.00025829110487652,0.000327654633621028,0.000399363990848623,
0.000469709285209461,0.000516310576520755),.UNSPECIFIED.);
#4266=B_SPLINE_CURVE_WITH_KNOTS('',3,(#168184,#168185,#168186,#168187,#168188,
#168189,#168190,#168191,#168192,#168193,#168194,#168195,#168196,#168197,
#168198,#168199,#168200,#168201,#168202,#168203,#168204,#168205,#168206,
#168207,#168208,#168209,#168210,#168211,#168212,#168213,#168214,#168215,
#168216,#168217,#168218,#168219,#168220,#168221,#168222,#168223),
 .UNSPECIFIED.,.F.,.F.,(4,3,3,3,3,3,3,3,3,3,3,3,3,4),(0.,6.84564250797382E-5,
0.000138288406590481,0.000205407478923822,0.00025696602122586,0.000257101146970262,
0.000271589374668168,0.000352213067609828,0.000388398097499862,0.000404123622054945,
0.000459162957997734,0.000486682625969129,0.000500442459954826,0.000514202293940523),
 .UNSPECIFIED.);
#4267=B_SPLINE_CURVE_WITH_KNOTS('',3,(#168227,#168228,#168229,#168230,#168231,
#168232,#168233,#168234,#168235,#168236,#168237,#168238,#168239,#168240,
#168241,#168242,#168243,#168244,#168245,#168246,#168247,#168248,#168249,
#168250,#168251,#168252,#168253,#168254,#168255,#168256,#168257,#168258,
#168259,#168260,#168261,#168262,#168263,#168264,#168265,#168266,#168267,
#168268,#168269),.UNSPECIFIED.,.F.,.F.,(4,3,3,3,3,3,3,3,3,3,3,3,3,3,4),
(0.,1.12890698065866E-5,7.65259667026273E-5,0.000102837507928552,0.000112544869199291,
0.000130746171581927,0.000194450729921151,0.000226303009090764,0.00024222914867557,
0.000258155288260376,0.000258291104876516,0.000327654633619408,0.000399363990846113,
0.000469709285207155,0.000516310576520752),.UNSPECIFIED.);
#4268=B_SPLINE_CURVE_WITH_KNOTS('',3,(#168277,#168278,#168279,#168280,#168281,
#168282,#168283,#168284,#168285,#168286,#168287,#168288,#168289,#168290,
#168291,#168292,#168293,#168294,#168295,#168296,#168297,#168298,#168299,
#168300,#168301,#168302,#168303,#168304,#168305,#168306,#168307,#168308,
#168309,#168310,#168311,#168312,#168313,#168314,#168315,#168316),
 .UNSPECIFIED.,.F.,.F.,(4,3,3,3,3,3,3,3,3,3,3,3,3,4),(0.,6.84564250840846E-5,
0.000138288406599155,0.00020540747893674,0.000256966021225868,0.000257101146970265,
0.000271589374668158,0.000352213067593023,0.000388398097499727,0.000404123622054827,
0.000459162957997679,0.000486682625969105,0.000500442459954818,0.000514202293940531),
 .UNSPECIFIED.);
#4269=B_SPLINE_CURVE_WITH_KNOTS('',3,(#168320,#168321,#168322,#168323,#168324,
#168325,#168326,#168327,#168328,#168329,#168330,#168331,#168332,#168333,
#168334,#168335,#168336,#168337,#168338,#168339,#168340,#168341,#168342,
#168343,#168344,#168345,#168346,#168347,#168348,#168349,#168350,#168351,
#168352,#168353,#168354,#168355,#168356,#168357,#168358,#168359,#168360,
#168361,#168362),.UNSPECIFIED.,.F.,.F.,(4,3,3,3,3,3,3,3,3,3,3,3,3,3,4),
(0.,1.12890698065756E-5,7.65259666974363E-5,0.000102837507928435,0.000112544869199181,
0.000130746171581831,0.000194450729921105,0.000226303009090742,0.00024222914867556,
0.000258155288260379,0.000258291104876533,0.000327654633620618,0.000399363990848227,
0.000469709285210271,0.000516310576520758),.UNSPECIFIED.);
#4270=B_SPLINE_CURVE_WITH_KNOTS('',3,(#168370,#168371,#168372,#168373,#168374,
#168375,#168376,#168377,#168378,#168379,#168380,#168381,#168382,#168383,
#168384,#168385,#168386,#168387,#168388,#168389,#168390,#168391,#168392,
#168393,#168394,#168395,#168396,#168397,#168398,#168399,#168400,#168401,
#168402,#168403,#168404,#168405,#168406,#168407,#168408,#168409),
 .UNSPECIFIED.,.F.,.F.,(4,3,3,3,3,3,3,3,3,3,3,3,3,4),(0.,6.84564250769302E-5,
0.000138288406583924,0.000205407478911775,0.000256966021225856,0.000257101146970262,
0.000271589374668158,0.000352213067622837,0.000388398097499689,0.000404123622054793,
0.000459162957997659,0.000486682625969092,0.000500442459954808,0.000514202293940524),
 .UNSPECIFIED.);
#4271=B_SPLINE_CURVE_WITH_KNOTS('',3,(#168413,#168414,#168415,#168416,#168417,
#168418,#168419,#168420,#168421,#168422,#168423,#168424,#168425,#168426,
#168427,#168428,#168429,#168430,#168431,#168432,#168433,#168434,#168435,
#168436,#168437,#168438,#168439,#168440,#168441,#168442,#168443,#168444,
#168445,#168446,#168447,#168448,#168449,#168450,#168451,#168452,#168453,
#168454,#168455),.UNSPECIFIED.,.F.,.F.,(4,3,3,3,3,3,3,3,3,3,3,3,3,3,4),
(0.,1.12890698065816E-5,7.65259666866503E-5,0.000102837507928537,0.000112544869199277,
0.000130746171581913,0.000194450729921141,0.000226303009090755,0.000242229148675562,
0.000258155288260369,0.000258291104876509,0.00032765463362347,0.000399363990852578,
0.000469709285214009,0.000516310576520738),.UNSPECIFIED.);
#4272=B_SPLINE_CURVE_WITH_KNOTS('',3,(#168463,#168464,#168465,#168466,#168467,
#168468,#168469,#168470,#168471,#168472,#168473,#168474,#168475,#168476,
#168477,#168478,#168479,#168480,#168481,#168482,#168483,#168484,#168485,
#168486,#168487,#168488,#168489,#168490,#168491,#168492,#168493,#168494,
#168495,#168496,#168497,#168498,#168499,#168500,#168501,#168502),
 .UNSPECIFIED.,.F.,.F.,(4,3,3,3,3,3,3,3,3,3,3,3,3,4),(0.,6.845642508705E-5,
0.000138288406605506,0.000205407478946818,0.000256966021225846,0.000257101146970255,
0.00027158937466815,0.00035221306759162,0.000388398097499678,0.000404123622054782,
0.000459162957997647,0.000486682625969079,0.000500442459954795,0.000514202293940511),
 .UNSPECIFIED.);
#4273=B_SPLINE_CURVE_WITH_KNOTS('',3,(#168506,#168507,#168508,#168509,#168510,
#168511,#168512,#168513,#168514,#168515,#168516,#168517,#168518,#168519,
#168520,#168521,#168522,#168523,#168524,#168525,#168526,#168527,#168528,
#168529,#168530,#168531,#168532,#168533,#168534,#168535,#168536,#168537,
#168538,#168539,#168540,#168541,#168542,#168543,#168544,#168545,#168546,
#168547,#168548),.UNSPECIFIED.,.F.,.F.,(4,3,3,3,3,3,3,3,3,3,3,3,3,3,4),
(0.,1.12890698065805E-5,7.65259667089018E-5,0.000102837507928513,0.000112544869199254,
0.000130746171581893,0.000194450729921131,0.00022630300909075,0.000242229148675559,
0.000258155288260369,0.00025829110487651,0.000327654633617099,0.000399363990841473,
0.000469709285200287,0.000516310576520737),.UNSPECIFIED.);
#4274=B_SPLINE_CURVE_WITH_KNOTS('',3,(#168556,#168557,#168558,#168559,#168560,
#168561,#168562,#168563,#168564,#168565,#168566,#168567,#168568,#168569,
#168570,#168571,#168572,#168573,#168574,#168575,#168576,#168577,#168578,
#168579,#168580,#168581,#168582,#168583,#168584,#168585,#168586,#168587,
#168588,#168589,#168590,#168591,#168592,#168593,#168594,#168595),
 .UNSPECIFIED.,.F.,.F.,(4,3,3,3,3,3,3,3,3,3,3,3,3,4),(0.,6.84564250895596E-5,
0.000138288406609849,0.000205407478950599,0.000256966021225854,0.000257101146970263,
0.000271589374668168,0.000352213067611649,0.000388398097499792,0.000404123622054883,
0.000459162957997705,0.000486682625969115,0.00050044245995482,0.000514202293940526),
 .UNSPECIFIED.);
#4275=B_SPLINE_CURVE_WITH_KNOTS('',3,(#168599,#168600,#168601,#168602,#168603,
#168604,#168605,#168606,#168607,#168608,#168609,#168610,#168611,#168612,
#168613,#168614,#168615,#168616,#168617,#168618,#168619,#168620,#168621,
#168622,#168623,#168624,#168625,#168626,#168627,#168628,#168629,#168630,
#168631,#168632,#168633,#168634,#168635,#168636,#168637,#168638,#168639,
#168640,#168641),.UNSPECIFIED.,.F.,.F.,(4,3,3,3,3,3,3,3,3,3,3,3,3,3,4),
(0.,1.12890698065891E-5,7.65259667078449E-5,0.000102837507928607,0.000112544869199342,
0.000130746171581971,0.000194450729921172,0.000226303009090772,0.000242229148675572,
0.000258155288260373,0.000258291104876515,0.000327654633617038,0.000399363990840811,
0.000469709285198597,0.000516310576520745),.UNSPECIFIED.);
#4276=B_SPLINE_CURVE_WITH_KNOTS('',3,(#168649,#168650,#168651,#168652,#168653,
#168654,#168655,#168656,#168657,#168658,#168659,#168660,#168661,#168662,
#168663,#168664,#168665,#168666,#168667,#168668,#168669,#168670,#168671,
#168672,#168673,#168674,#168675,#168676,#168677,#168678,#168679,#168680,
#168681,#168682,#168683,#168684,#168685,#168686,#168687,#168688),
 .UNSPECIFIED.,.F.,.F.,(4,3,3,3,3,3,3,3,3,3,3,3,3,4),(0.,6.84564250838755E-5,
0.000138288406598415,0.00020540747893465,0.000256966021225841,0.000257101146970261,
0.000271589374668164,0.0003522130676064,0.000388398097499832,0.000404123622054918,
0.000459162957997721,0.000486682625969122,0.000500442459954822,0.000514202293940523),
 .UNSPECIFIED.);
#4277=B_SPLINE_CURVE_WITH_KNOTS('',3,(#168692,#168693,#168694,#168695,#168696,
#168697,#168698,#168699,#168700,#168701,#168702,#168703,#168704,#168705,
#168706,#168707,#168708,#168709,#168710,#168711,#168712,#168713,#168714,
#168715,#168716,#168717,#168718,#168719,#168720,#168721,#168722,#168723,
#168724,#168725,#168726,#168727,#168728,#168729,#168730,#168731,#168732,
#168733,#168734),.UNSPECIFIED.,.F.,.F.,(4,3,3,3,3,3,3,3,3,3,3,3,3,3,4),
(0.,1.12890698065788E-5,7.65259667132543E-5,0.000102837507928489,0.000112544869199232,
0.000130746171581874,0.000194450729921125,0.00022630300909075,0.000242229148675562,
0.000258155288260375,0.000258291104876516,0.000327654633612138,0.000399363990830831,
0.000469709285183981,0.00051631057652075),.UNSPECIFIED.);
#4278=B_SPLINE_CURVE_WITH_KNOTS('',3,(#168742,#168743,#168744,#168745,#168746,
#168747,#168748,#168749,#168750,#168751,#168752,#168753,#168754,#168755,
#168756,#168757,#168758,#168759,#168760,#168761,#168762,#168763,#168764,
#168765,#168766,#168767,#168768,#168769,#168770,#168771,#168772,#168773,
#168774,#168775,#168776,#168777,#168778,#168779,#168780,#168781),
 .UNSPECIFIED.,.F.,.F.,(4,3,3,3,3,3,3,3,3,3,3,3,3,4),(0.,6.84564250765995E-5,
0.000138288406584294,0.000205407478915326,0.000256966021225849,0.000257101146970262,
0.000271589374668161,0.000352213067601591,0.000388398097499769,0.000404123622054863,
0.000459162957997693,0.000486682625969109,0.000500442459954816,0.000514202293940524),
 .UNSPECIFIED.);
#4279=B_SPLINE_CURVE_WITH_KNOTS('',3,(#168785,#168786,#168787,#168788,#168789,
#168790,#168791,#168792,#168793,#168794,#168795,#168796,#168797,#168798,
#168799,#168800,#168801,#168802,#168803,#168804,#168805,#168806,#168807,
#168808,#168809,#168810,#168811,#168812,#168813,#168814,#168815,#168816,
#168817,#168818,#168819,#168820,#168821,#168822,#168823,#168824,#168825,
#168826,#168827),.UNSPECIFIED.,.F.,.F.,(4,3,3,3,3,3,3,3,3,3,3,3,3,3,4),
(3.46944695195361E-18,1.12890698065869E-5,7.65259667025008E-5,0.000102837507928517,
0.000112544869199258,0.000130746171581898,0.000194450729921137,0.000226303009090756,
0.000242229148675566,0.000258155288260376,0.000258291104876511,0.000327654633609564,
0.000399363990824879,0.000469709285174596,0.000516310576520748),
 .UNSPECIFIED.);
#4280=B_SPLINE_CURVE_WITH_KNOTS('',3,(#168835,#168836,#168837,#168838,#168839,
#168840,#168841,#168842,#168843,#168844,#168845,#168846,#168847,#168848,
#168849,#168850,#168851,#168852,#168853,#168854,#168855,#168856,#168857,
#168858,#168859,#168860,#168861,#168862,#168863,#168864,#168865,#168866,
#168867,#168868,#168869,#168870,#168871,#168872,#168873,#168874),
 .UNSPECIFIED.,.F.,.F.,(4,3,3,3,3,3,3,3,3,3,3,3,3,4),(0.,6.84564250797669E-5,
0.000138288406590498,0.000205407478924127,0.000256966021225838,0.000257101146970264,
0.000271589374668166,0.000352213067600068,0.000388398097499821,0.00040412362205491,
0.000459162957997718,0.000486682625969123,0.000500442459954825,0.000514202293940527),
 .UNSPECIFIED.);
#4281=B_SPLINE_CURVE_WITH_KNOTS('',3,(#168878,#168879,#168880,#168881,#168882,
#168883,#168884,#168885,#168886,#168887,#168888,#168889,#168890,#168891,
#168892,#168893,#168894,#168895,#168896,#168897,#168898,#168899,#168900,
#168901,#168902,#168903,#168904,#168905,#168906,#168907,#168908,#168909,
#168910,#168911,#168912,#168913,#168914,#168915,#168916,#168917,#168918,
#168919,#168920),.UNSPECIFIED.,.F.,.F.,(4,3,3,3,3,3,3,3,3,3,3,3,3,3,4),
(1.73472347597681E-18,1.12890698065832E-5,7.65259667045979E-5,0.000102837507928536,
0.000112544869199276,0.000130746171581912,0.00019445072992114,0.000226303009090754,
0.000242229148675561,0.000258155288260368,0.000258291104876511,0.000327654633615822,
0.000399363990838075,0.000469709285194198,0.000516310576520735),
 .UNSPECIFIED.);
#4282=B_SPLINE_CURVE_WITH_KNOTS('',3,(#168928,#168929,#168930,#168931,#168932,
#168933,#168934,#168935,#168936,#168937,#168938,#168939,#168940,#168941,
#168942,#168943,#168944,#168945,#168946,#168947,#168948,#168949,#168950,
#168951,#168952,#168953,#168954,#168955,#168956,#168957,#168958,#168959,
#168960,#168961,#168962,#168963,#168964,#168965,#168966,#168967),
 .UNSPECIFIED.,.F.,.F.,(4,3,3,3,3,3,3,3,3,3,3,3,3,4),(0.,6.84564250822334E-5,
0.000138288406595693,0.000205407478931659,0.000256966021225854,0.000257101146970264,
0.000271589374668166,0.000352213067615386,0.000388398097499783,0.000404123622054876,
0.000459162957997701,0.000486682625969114,0.000500442459954821,0.000514202293940527),
 .UNSPECIFIED.);
#4283=B_SPLINE_CURVE_WITH_KNOTS('',3,(#168971,#168972,#168973,#168974,#168975,
#168976,#168977,#168978,#168979,#168980,#168981,#168982,#168983,#168984,
#168985,#168986,#168987,#168988,#168989,#168990,#168991,#168992,#168993,
#168994,#168995,#168996,#168997,#168998,#168999,#169000,#169001,#169002,
#169003,#169004,#169005,#169006,#169007,#169008,#169009,#169010,#169011,
#169012,#169013),.UNSPECIFIED.,.F.,.F.,(4,3,3,3,3,3,3,3,3,3,3,3,3,3,4),
(0.,1.12890698065817E-5,7.652596670597E-5,0.000102837507928492,0.000112544869199235,
0.000130746171581877,0.000194450729921126,0.00022630300909075,0.000242229148675562,
0.000258155288260375,0.000258291104876527,0.000327654633612159,0.000399363990830566,
0.000469709285183404,0.000516310576520749),.UNSPECIFIED.);
#4284=B_SPLINE_CURVE_WITH_KNOTS('',3,(#169021,#169022,#169023,#169024,#169025,
#169026,#169027,#169028,#169029,#169030,#169031,#169032,#169033,#169034,
#169035,#169036,#169037,#169038,#169039,#169040,#169041,#169042,#169043,
#169044,#169045,#169046,#169047,#169048,#169049,#169050,#169051,#169052,
#169053,#169054,#169055,#169056,#169057,#169058,#169059,#169060),
 .UNSPECIFIED.,.F.,.F.,(4,3,3,3,3,3,3,3,3,3,3,3,3,4),(0.,6.84564250761049E-5,
0.00013828840658303,0.000205407478912784,0.000256966021225849,0.000257101146970261,
0.000271589374668167,0.000352213067604775,0.000388398097499802,0.000404123622054892,
0.000459162957997707,0.000486682625969115,0.000500442459954818,0.000514202293940522),
 .UNSPECIFIED.);
#4285=B_SPLINE_CURVE_WITH_KNOTS('',3,(#169064,#169065,#169066,#169067,#169068,
#169069,#169070,#169071,#169072,#169073,#169074,#169075,#169076,#169077,
#169078,#169079,#169080,#169081,#169082,#169083,#169084,#169085,#169086,
#169087,#169088,#169089,#169090,#169091,#169092,#169093,#169094,#169095,
#169096,#169097,#169098,#169099,#169100,#169101,#169102,#169103,#169104,
#169105,#169106),.UNSPECIFIED.,.F.,.F.,(4,3,3,3,3,3,3,3,3,3,3,3,3,3,4),
(0.,1.12890698065779E-5,7.65259667127145E-5,0.000102837507928481,0.000112544869199224,
0.000130746171581867,0.000194450729921117,0.000226303009090742,0.000242229148675555,
0.000258155288260368,0.000258291104876507,0.000327654633610104,0.000399363990826758,
0.000469709285178193,0.000516310576520735),.UNSPECIFIED.);
#4286=B_SPLINE_CURVE_WITH_KNOTS('',3,(#169114,#169115,#169116,#169117,#169118,
#169119,#169120,#169121,#169122,#169123,#169124,#169125,#169126,#169127,
#169128,#169129,#169130,#169131,#169132,#169133,#169134,#169135,#169136,
#169137,#169138,#169139,#169140,#169141,#169142,#169143,#169144,#169145,
#169146,#169147,#169148,#169149,#169150,#169151,#169152,#169153),
 .UNSPECIFIED.,.F.,.F.,(4,3,3,3,3,3,3,3,3,3,3,3,3,4),(0.,6.84564250890086E-5,
0.000138288406609153,0.000205407478951144,0.000256966021225856,0.000257101146970263,
0.000271589374668163,0.00035221306760415,0.000388398097499778,0.000404123622054872,
0.000459162957997699,0.000486682625969112,0.000500442459954819,0.000514202293940526),
 .UNSPECIFIED.);
#4287=B_SPLINE_CURVE_WITH_KNOTS('',3,(#169157,#169158,#169159,#169160,#169161,
#169162,#169163,#169164,#169165,#169166,#169167,#169168,#169169,#169170,
#169171,#169172,#169173,#169174,#169175,#169176,#169177,#169178,#169179,
#169180,#169181,#169182,#169183,#169184,#169185,#169186,#169187,#169188,
#169189,#169190,#169191,#169192,#169193,#169194,#169195,#169196,#169197,
#169198,#169199),.UNSPECIFIED.,.F.,.F.,(4,3,3,3,3,3,3,3,3,3,3,3,3,3,4),
(8.67361737988404E-19,1.12890698065823E-5,7.65259666978494E-5,0.000102837507928528,
0.000112544869199268,0.000130746171581906,0.000194450729921138,0.000226303009090754,
0.000242229148675562,0.000258155288260371,0.0002582911048765,0.000327654633618696,
0.000399363990843831,0.000469709285202593,0.00051631057652074),
 .UNSPECIFIED.);
#4288=B_SPLINE_CURVE_WITH_KNOTS('',3,(#169207,#169208,#169209,#169210,#169211,
#169212,#169213,#169214,#169215,#169216,#169217,#169218,#169219,#169220,
#169221,#169222,#169223,#169224,#169225,#169226,#169227,#169228,#169229,
#169230,#169231,#169232,#169233,#169234,#169235,#169236,#169237,#169238,
#169239,#169240,#169241,#169242,#169243,#169244,#169245,#169246),
 .UNSPECIFIED.,.F.,.F.,(4,3,3,3,3,3,3,3,3,3,3,3,3,4),(0.,6.84564250864531E-5,
0.000138288406604524,0.000205407478945309,0.000256966021225842,0.000257101146970264,
0.000271589374668167,0.00035221306760789,0.000388398097499815,0.000404123622054904,
0.000459162957997716,0.000486682625969122,0.000500442459954825,0.000514202293940528),
 .UNSPECIFIED.);
#4289=B_SPLINE_CURVE_WITH_KNOTS('',3,(#169250,#169251,#169252,#169253,#169254,
#169255,#169256,#169257,#169258,#169259,#169260,#169261,#169262,#169263,
#169264,#169265,#169266,#169267,#169268,#169269,#169270,#169271,#169272,
#169273,#169274,#169275,#169276,#169277,#169278,#169279,#169280,#169281,
#169282,#169283,#169284,#169285,#169286,#169287,#169288,#169289,#169290,
#169291,#169292),.UNSPECIFIED.,.F.,.F.,(4,3,3,3,3,3,3,3,3,3,3,3,3,3,4),
(1.73472347597681E-18,1.12890698065862E-5,7.652596670712E-5,0.000102837507928532,
0.000112544869199272,0.000130746171581909,0.000194450729921137,0.000226303009090752,
0.000242229148675559,0.000258155288260366,0.000258291104876512,0.000327654633614979,
0.000399363990836396,0.000469709285192041,0.00051631057652073),
 .UNSPECIFIED.);
#4290=B_SPLINE_CURVE_WITH_KNOTS('',3,(#169300,#169301,#169302,#169303,#169304,
#169305,#169306,#169307,#169308,#169309,#169310,#169311,#169312,#169313,
#169314,#169315,#169316,#169317,#169318,#169319,#169320,#169321,#169322,
#169323,#169324,#169325,#169326,#169327,#169328,#169329,#169330,#169331,
#169332,#169333,#169334,#169335,#169336,#169337,#169338,#169339),
 .UNSPECIFIED.,.F.,.F.,(4,3,3,3,3,3,3,3,3,3,3,3,3,4),(0.,6.84564250871121E-5,
0.000138288406605608,0.000205407478946803,0.000256966021225858,0.000257101146970267,
0.000271589374668171,0.000352213067596241,0.000388398097499807,0.000404123622054898,
0.000459162957997716,0.000486682625969125,0.000500442459954829,0.000514202293940534),
 .UNSPECIFIED.);
#4291=B_SPLINE_CURVE_WITH_KNOTS('',3,(#169343,#169344,#169345,#169346,#169347,
#169348,#169349,#169350,#169351,#169352,#169353,#169354,#169355,#169356,
#169357,#169358,#169359,#169360,#169361,#169362,#169363,#169364,#169365,
#169366,#169367,#169368,#169369,#169370,#169371,#169372,#169373,#169374,
#169375,#169376,#169377,#169378,#169379,#169380,#169381,#169382,#169383,
#169384,#169385),.UNSPECIFIED.,.F.,.F.,(4,3,3,3,3,3,3,3,3,3,3,3,3,3,4),
(0.,1.12890698065804E-5,7.65259666985084E-5,0.000102837507928506,0.000112544869199248,
0.000130746171581889,0.000194450729921132,0.000226303009090753,0.000242229148675564,
0.000258155288260375,0.000258291104876532,0.000327654633619549,0.000399363990845382,
0.000469709285204578,0.00051631057652075),.UNSPECIFIED.);
#4292=B_SPLINE_CURVE_WITH_KNOTS('',3,(#169393,#169394,#169395,#169396,#169397,
#169398,#169399,#169400,#169401,#169402,#169403,#169404,#169405,#169406,
#169407,#169408,#169409,#169410,#169411,#169412,#169413,#169414,#169415,
#169416,#169417,#169418,#169419,#169420,#169421,#169422,#169423,#169424,
#169425,#169426,#169427,#169428,#169429,#169430,#169431,#169432),
 .UNSPECIFIED.,.F.,.F.,(4,3,3,3,3,3,3,3,3,3,3,3,3,4),(0.,6.84564250843184E-5,
0.000138288406599641,0.000205407478937078,0.000256966021225852,0.000257101146970261,
0.000271589374668166,0.000352213067604727,0.000388398097499781,0.000404123622054874,
0.000459162957997697,0.000486682625969109,0.000500442459954815,0.000514202293940521),
 .UNSPECIFIED.);
#4293=B_SPLINE_CURVE_WITH_KNOTS('',3,(#169436,#169437,#169438,#169439,#169440,
#169441,#169442,#169443,#169444,#169445,#169446,#169447,#169448,#169449,
#169450,#169451,#169452,#169453,#169454,#169455,#169456,#169457,#169458,
#169459,#169460,#169461,#169462,#169463,#169464,#169465,#169466,#169467,
#169468,#169469,#169470,#169471,#169472,#169473,#169474,#169475,#169476,
#169477,#169478),.UNSPECIFIED.,.F.,.F.,(4,3,3,3,3,3,3,3,3,3,3,3,3,3,4),
(0.,1.12890698065816E-5,7.65259667114556E-5,0.000102837507928525,0.000112544869199266,
0.000130746171581904,0.00019445072992114,0.000226303009090757,0.000242229148675566,
0.000258155288260375,0.000258291104876523,0.00032765463361819,0.000399363990843023,
0.000469709285201166,0.000516310576520736),.UNSPECIFIED.);
#4294=B_SPLINE_CURVE_WITH_KNOTS('',3,(#169486,#169487,#169488,#169489,#169490,
#169491,#169492,#169493,#169494,#169495,#169496,#169497,#169498,#169499,
#169500,#169501,#169502,#169503,#169504,#169505,#169506,#169507,#169508,
#169509,#169510,#169511,#169512,#169513,#169514,#169515,#169516,#169517,
#169518,#169519,#169520,#169521,#169522,#169523,#169524,#169525),
 .UNSPECIFIED.,.F.,.F.,(4,3,3,3,3,3,3,3,3,3,3,3,3,4),(0.,6.8456425074579E-5,
0.000138288406580344,0.000205407478909642,0.000256966021225861,0.000257101146970265,
0.00027158937466816,0.000352213067612298,0.000388398097499719,0.00040412362205482,
0.000459162957997671,0.000486682625969096,0.000500442459954809,0.000514202293940522),
 .UNSPECIFIED.);
#4295=B_SPLINE_CURVE_WITH_KNOTS('',3,(#169529,#169530,#169531,#169532,#169533,
#169534,#169535,#169536,#169537,#169538,#169539,#169540,#169541,#169542,
#169543,#169544,#169545,#169546,#169547,#169548,#169549,#169550,#169551,
#169552,#169553,#169554,#169555,#169556,#169557,#169558,#169559,#169560,
#169561,#169562,#169563,#169564,#169565,#169566,#169567,#169568,#169569,
#169570,#169571),.UNSPECIFIED.,.F.,.F.,(4,3,3,3,3,3,3,3,3,3,3,3,3,3,4),
(0.,1.12890698065828E-5,7.6525966717577E-5,0.000102837507928482,0.000112544869199225,
0.000130746171581869,0.000194450729921122,0.000226303009090749,0.000242229148675563,
0.000258155288260376,0.000258291104876513,0.000327654633621626,0.000399363990850335,
0.000469709285212286,0.000516310576520752),.UNSPECIFIED.);
#4296=B_SPLINE_CURVE_WITH_KNOTS('',3,(#169579,#169580,#169581,#169582,#169583,
#169584,#169585,#169586,#169587,#169588,#169589,#169590,#169591,#169592,
#169593,#169594,#169595,#169596,#169597,#169598,#169599,#169600,#169601,
#169602,#169603,#169604,#169605,#169606,#169607,#169608,#169609,#169610,
#169611,#169612,#169613,#169614,#169615,#169616,#169617,#169618),
 .UNSPECIFIED.,.F.,.F.,(4,3,3,3,3,3,3,3,3,3,3,3,3,4),(0.,6.84564250758689E-5,
0.000138288406581853,0.000205407478909165,0.000256966021225856,0.00025710114697026,
0.000271589374668164,0.00035221306760689,0.000388398097499763,0.000404123622054857,
0.000459162957997689,0.000486682625969104,0.000500442459954812,0.00051420229394052),
 .UNSPECIFIED.);
#4297=B_SPLINE_CURVE_WITH_KNOTS('',3,(#169622,#169623,#169624,#169625,#169626,
#169627,#169628,#169629,#169630,#169631,#169632,#169633,#169634,#169635,
#169636,#169637,#169638,#169639,#169640,#169641,#169642,#169643,#169644,
#169645,#169646,#169647,#169648,#169649,#169650,#169651,#169652,#169653,
#169654,#169655,#169656,#169657,#169658,#169659,#169660,#169661,#169662,
#169663,#169664),.UNSPECIFIED.,.F.,.F.,(4,3,3,3,3,3,3,3,3,3,3,3,3,3,4),
(0.,1.12890698065862E-5,7.65259667010518E-5,0.000102837507928541,0.00011254486919928,
0.000130746171581917,0.000194450729921143,0.000226303009090756,0.000242229148675563,
0.000258155288260369,0.000258291104876529,0.000327654633612457,0.000399363990831282,
0.000469709285184427,0.000516310576520739),.UNSPECIFIED.);
#4298=B_SPLINE_CURVE_WITH_KNOTS('',3,(#169672,#169673,#169674,#169675,#169676,
#169677,#169678,#169679,#169680,#169681,#169682,#169683,#169684,#169685,
#169686,#169687,#169688,#169689,#169690,#169691,#169692,#169693,#169694,
#169695,#169696,#169697,#169698,#169699,#169700,#169701,#169702,#169703,
#169704,#169705,#169706,#169707,#169708,#169709,#169710,#169711),
 .UNSPECIFIED.,.F.,.F.,(4,3,3,3,3,3,3,3,3,3,3,3,3,4),(0.,6.84564250843761E-5,
0.000138288406600102,0.000205407478938898,0.00025696602122586,0.000257101146970268,
0.000271589374668179,0.000352213067592679,0.000388398097499883,0.000404123622054964,
0.00045916295799775,0.000486682625969143,0.000500442459954839,0.000514202293940536),
 .UNSPECIFIED.);
#4299=B_SPLINE_CURVE_WITH_KNOTS('',3,(#169715,#169716,#169717,#169718,#169719,
#169720,#169721,#169722,#169723,#169724,#169725,#169726,#169727,#169728,
#169729,#169730,#169731,#169732,#169733,#169734,#169735,#169736,#169737,
#169738,#169739,#169740,#169741,#169742,#169743,#169744,#169745,#169746,
#169747,#169748,#169749,#169750,#169751,#169752,#169753,#169754,#169755,
#169756,#169757),.UNSPECIFIED.,.F.,.F.,(4,3,3,3,3,3,3,3,3,3,3,3,3,3,4),
(0.,1.12890698065796E-5,7.65259666991178E-5,0.000102837507928466,0.000112544869199211,
0.000130746171581857,0.000194450729921119,0.000226303009090749,0.000242229148675565,
0.00025815528826038,0.000258291104876507,0.000327654633623256,0.000399363990854542,
0.000469709285220818,0.000516310576520761),.UNSPECIFIED.);
#4300=B_SPLINE_CURVE_WITH_KNOTS('',3,(#169765,#169766,#169767,#169768,#169769,
#169770,#169771,#169772,#169773,#169774,#169775,#169776,#169777,#169778,
#169779,#169780,#169781,#169782,#169783,#169784,#169785,#169786,#169787,
#169788,#169789,#169790,#169791,#169792,#169793,#169794,#169795,#169796,
#169797,#169798,#169799,#169800,#169801,#169802,#169803,#169804),
 .UNSPECIFIED.,.F.,.F.,(4,3,3,3,3,3,3,3,3,3,3,3,3,4),(0.,6.8456425090809E-5,
0.000138288406613196,0.00020540747895784,0.000256966021225841,0.000257101146970264,
0.000271589374668169,0.000352213067601343,0.000388398097499806,0.000404123622054896,
0.000459162957997712,0.00048668262596912,0.000500442459954824,0.000514202293940528),
 .UNSPECIFIED.);
#4301=B_SPLINE_CURVE_WITH_KNOTS('',3,(#169808,#169809,#169810,#169811,#169812,
#169813,#169814,#169815,#169816,#169817,#169818,#169819,#169820,#169821,
#169822,#169823,#169824,#169825,#169826,#169827,#169828,#169829,#169830,
#169831,#169832,#169833,#169834,#169835,#169836,#169837,#169838,#169839,
#169840,#169841,#169842,#169843,#169844,#169845,#169846,#169847,#169848,
#169849,#169850),.UNSPECIFIED.,.F.,.F.,(4,3,3,3,3,3,3,3,3,3,3,3,3,3,4),
(0.,1.12890698065837E-5,7.65259666927835E-5,0.000102837507928546,0.000112544869199286,
0.000130746171581922,0.000194450729921148,0.000226303009090761,0.000242229148675567,
0.000258155288260374,0.000258291104876513,0.000327654633617415,0.000399363990840611,
0.000469709285196912,0.000516310576520748),.UNSPECIFIED.);
#4302=B_SPLINE_CURVE_WITH_KNOTS('',3,(#169858,#169859,#169860,#169861,#169862,
#169863,#169864,#169865,#169866,#169867,#169868,#169869,#169870,#169871,
#169872,#169873,#169874,#169875,#169876,#169877,#169878,#169879,#169880,
#169881,#169882,#169883,#169884,#169885,#169886,#169887,#169888,#169889,
#169890,#169891,#169892,#169893,#169894,#169895,#169896,#169897),
 .UNSPECIFIED.,.F.,.F.,(4,3,3,3,3,3,3,3,3,3,3,3,3,4),(0.,6.84564250857982E-5,
0.000138288406602572,0.000205407478941416,0.000256966021225879,0.000257101146970264,
0.000271589374668177,0.000352213067604349,0.000388398097499876,0.000404123622054957,
0.000459162957997742,0.000486682625969135,0.000500442459954831,0.000514202293940528),
 .UNSPECIFIED.);
#4303=B_SPLINE_CURVE_WITH_KNOTS('',3,(#169901,#169902,#169903,#169904,#169905,
#169906,#169907,#169908,#169909,#169910,#169911,#169912,#169913,#169914,
#169915,#169916,#169917,#169918,#169919,#169920,#169921,#169922,#169923,
#169924,#169925,#169926,#169927,#169928,#169929,#169930,#169931,#169932,
#169933,#169934,#169935,#169936,#169937,#169938,#169939,#169940,#169941,
#169942,#169943),.UNSPECIFIED.,.F.,.F.,(4,3,3,3,3,3,3,3,3,3,3,3,3,3,4),
(0.,1.12890698065829E-5,7.6525966704634E-5,0.00010283750792853,0.000112544869199271,
0.000130746171581909,0.000194450729921141,0.000226303009090758,0.000242229148675566,
0.000258155288260374,0.000258291104876519,0.000327654633610232,0.000399363990826456,
0.000469709285177114,0.000516310576520749),.UNSPECIFIED.);
#4304=B_SPLINE_CURVE_WITH_KNOTS('',3,(#169951,#169952,#169953,#169954,#169955,
#169956,#169957,#169958,#169959,#169960,#169961,#169962,#169963,#169964,
#169965,#169966,#169967,#169968,#169969,#169970,#169971,#169972,#169973,
#169974,#169975,#169976,#169977,#169978,#169979,#169980,#169981,#169982,
#169983,#169984,#169985,#169986,#169987,#169988,#169989,#169990),
 .UNSPECIFIED.,.F.,.F.,(4,3,3,3,3,3,3,3,3,3,3,3,3,4),(0.,6.84564250862363E-5,
0.00013828840660365,0.000205407478943243,0.000256966021225853,0.000257101146970269,
0.000271589374668181,0.000352213067603087,0.000388398097499869,0.000404123622054952,
0.000459162957997745,0.000486682625969141,0.000500442459954839,0.000514202293940537),
 .UNSPECIFIED.);
#4305=B_SPLINE_CURVE_WITH_KNOTS('',3,(#169994,#169995,#169996,#169997,#169998,
#169999,#170000,#170001,#170002,#170003,#170004,#170005,#170006,#170007,
#170008,#170009,#170010,#170011,#170012,#170013,#170014,#170015,#170016,
#170017,#170018,#170019,#170020,#170021,#170022,#170023,#170024,#170025,
#170026,#170027,#170028,#170029,#170030,#170031,#170032,#170033,#170034,
#170035,#170036),.UNSPECIFIED.,.F.,.F.,(4,3,3,3,3,3,3,3,3,3,3,3,3,3,4),
(0.,1.12890698065816E-5,7.65259667227941E-5,0.000102837507928512,0.000112544869199253,
0.000130746171581893,0.000194450729921135,0.000226303009090755,0.000242229148675565,
0.000258155288260376,0.000258291104876516,0.000327654633614687,0.000399363990836629,
0.00046970928519338,0.000516310576520744),.UNSPECIFIED.);
#4306=B_SPLINE_CURVE_WITH_KNOTS('',3,(#170044,#170045,#170046,#170047,#170048,
#170049,#170050,#170051,#170052,#170053,#170054,#170055,#170056,#170057,
#170058,#170059,#170060,#170061,#170062,#170063,#170064,#170065,#170066,
#170067,#170068,#170069,#170070,#170071,#170072,#170073,#170074,#170075,
#170076,#170077,#170078,#170079,#170080,#170081,#170082,#170083),
 .UNSPECIFIED.,.F.,.F.,(4,3,3,3,3,3,3,3,3,3,3,3,3,4),(0.,6.84564250861885E-5,
0.000138288406603737,0.00020540747894416,0.000256966021225845,0.000257101146970264,
0.000271589374668171,0.000352213067589949,0.000388398097499864,0.000404123622054947,
0.000459162957997737,0.000486682625969132,0.00050044245995483,0.000514202293940528),
 .UNSPECIFIED.);
#4307=B_SPLINE_CURVE_WITH_KNOTS('',3,(#170087,#170088,#170089,#170090,#170091,
#170092,#170093,#170094,#170095,#170096,#170097,#170098,#170099,#170100,
#170101,#170102,#170103,#170104,#170105,#170106,#170107,#170108,#170109,
#170110,#170111,#170112,#170113,#170114,#170115,#170116,#170117,#170118,
#170119,#170120,#170121,#170122,#170123,#170124,#170125,#170126,#170127,
#170128,#170129),.UNSPECIFIED.,.F.,.F.,(4,3,3,3,3,3,3,3,3,3,3,3,3,3,4),
(0.,1.12890698065835E-5,7.65259666994345E-5,0.0001028375079285,0.000112544869199242,
0.000130746171581883,0.000194450729921126,0.000226303009090747,0.000242229148675558,
0.000258155288260369,0.00025829110487652,0.000327654633625233,0.000399363990857316,
0.000469709285222563,0.000516310576520737),.UNSPECIFIED.);
#4308=B_SPLINE_CURVE_WITH_KNOTS('',3,(#170137,#170138,#170139,#170140,#170141,
#170142,#170143,#170144,#170145,#170146,#170147,#170148,#170149,#170150,
#170151,#170152,#170153,#170154,#170155,#170156,#170157,#170158,#170159,
#170160,#170161,#170162,#170163,#170164,#170165,#170166,#170167,#170168,
#170169,#170170,#170171,#170172,#170173,#170174,#170175,#170176),
 .UNSPECIFIED.,.F.,.F.,(4,3,3,3,3,3,3,3,3,3,3,3,3,4),(0.,6.84564250829992E-5,
0.000138288406596676,0.000205407478932091,0.000256966021225855,0.000257101146970265,
0.000271589374668167,0.00035221306760733,0.000388398097499791,0.000404123622054884,
0.000459162957997707,0.000486682625969119,0.000500442459954825,0.000514202293940531),
 .UNSPECIFIED.);
#4309=B_SPLINE_CURVE_WITH_KNOTS('',3,(#170180,#170181,#170182,#170183,#170184,
#170185,#170186,#170187,#170188,#170189,#170190,#170191,#170192,#170193,
#170194,#170195,#170196,#170197,#170198,#170199,#170200,#170201,#170202,
#170203,#170204,#170205,#170206,#170207,#170208,#170209,#170210,#170211,
#170212,#170213,#170214,#170215,#170216,#170217,#170218,#170219,#170220,
#170221,#170222),.UNSPECIFIED.,.F.,.F.,(4,3,3,3,3,3,3,3,3,3,3,3,3,3,4),
(0.,1.12890698065865E-5,7.65259667007628E-5,0.000102837507928553,0.000112544869199292,
0.000130746171581927,0.000194450729921151,0.000226303009090763,0.000242229148675569,
0.000258155288260375,0.000258291104876515,0.000327654633620995,0.000399363990848543,
0.00046970928520939,0.00051631057652075),.UNSPECIFIED.);
#4310=B_SPLINE_CURVE_WITH_KNOTS('',3,(#170230,#170231,#170232,#170233,#170234,
#170235,#170236,#170237,#170238,#170239,#170240,#170241,#170242,#170243,
#170244,#170245,#170246,#170247,#170248,#170249,#170250,#170251,#170252,
#170253,#170254,#170255,#170256,#170257,#170258,#170259,#170260,#170261,
#170262,#170263,#170264,#170265,#170266,#170267,#170268,#170269),
 .UNSPECIFIED.,.F.,.F.,(4,3,3,3,3,3,3,3,3,3,3,3,3,4),(0.,6.84564250862226E-5,
0.000138288406603668,0.000205407478943698,0.00025696602122584,0.000257101146970262,
0.000271589374668167,0.000352213067598809,0.000388398097499793,0.000404123622054884,
0.000459162957997704,0.000486682625969114,0.000500442459954819,0.000514202293940524),
 .UNSPECIFIED.);
#4311=B_SPLINE_CURVE_WITH_KNOTS('',3,(#170273,#170274,#170275,#170276,#170277,
#170278,#170279,#170280,#170281,#170282,#170283,#170284,#170285,#170286,
#170287,#170288,#170289,#170290,#170291,#170292,#170293,#170294,#170295,
#170296,#170297,#170298,#170299,#170300,#170301,#170302,#170303,#170304,
#170305,#170306,#170307,#170308,#170309,#170310,#170311,#170312,#170313,
#170314,#170315),.UNSPECIFIED.,.F.,.F.,(4,3,3,3,3,3,3,3,3,3,3,3,3,3,4),
(0.,1.1289069806586E-5,7.65259667026302E-5,0.000102837507928521,0.000112544869199262,
0.000130746171581899,0.000194450729921131,0.000226303009090747,0.000242229148675555,
0.000258155288260363,0.000258291104876498,0.000327654633617347,0.000399363990841111,
0.000469709285198713,0.000516310576520727),.UNSPECIFIED.);
#4312=B_SPLINE_CURVE_WITH_KNOTS('',3,(#170323,#170324,#170325,#170326,#170327,
#170328,#170329,#170330,#170331,#170332,#170333,#170334,#170335,#170336,
#170337,#170338,#170339,#170340,#170341,#170342,#170343,#170344,#170345,
#170346,#170347,#170348,#170349,#170350,#170351,#170352,#170353,#170354,
#170355,#170356,#170357,#170358,#170359,#170360,#170361,#170362),
 .UNSPECIFIED.,.F.,.F.,(4,3,3,3,3,3,3,3,3,3,3,3,3,4),(0.,6.84564250893229E-5,
0.000138288406610045,0.000205407478953388,0.000256966021225841,0.000257101146970263,
0.00027158937466816,0.000352213067592389,0.000388398097499739,0.000404123622054837,
0.000459162957997681,0.000486682625969103,0.000500442459954814,0.000514202293940525),
 .UNSPECIFIED.);
#4313=B_SPLINE_CURVE_WITH_KNOTS('',3,(#170366,#170367,#170368,#170369,#170370,
#170371,#170372,#170373,#170374,#170375,#170376,#170377,#170378,#170379,
#170380,#170381,#170382,#170383,#170384,#170385,#170386,#170387,#170388,
#170389,#170390,#170391,#170392,#170393,#170394,#170395,#170396,#170397,
#170398,#170399,#170400,#170401,#170402,#170403,#170404,#170405,#170406,
#170407,#170408),.UNSPECIFIED.,.F.,.F.,(4,3,3,3,3,3,3,3,3,3,3,3,3,3,4),
(0.,1.12890698065853E-5,7.6525966706682E-5,0.000102837507928526,0.000112544869199267,
0.000130746171581906,0.000194450729921142,0.00022630300909076,0.000242229148675569,
0.000258155288260379,0.000258291104876522,0.000327654633611439,0.000399363990829307,
0.000469709285181712,0.000516310576520757),.UNSPECIFIED.);
#4314=B_SPLINE_CURVE_WITH_KNOTS('',3,(#170415,#170416,#170417,#170418,#170419,
#170420,#170421,#170422,#170423,#170424,#170425,#170426,#170427,#170428,
#170429,#170430,#170431,#170432,#170433,#170434,#170435,#170436,#170437,
#170438,#170439,#170440,#170441,#170442,#170443,#170444,#170445,#170446,
#170447,#170448,#170449,#170450,#170451,#170452,#170453,#170454),
 .UNSPECIFIED.,.F.,.F.,(4,3,3,3,3,3,3,3,3,3,3,3,3,4),(0.,6.84564250828479E-5,
0.000138288406596811,0.000205407478933446,0.000256966021225857,0.000257101146970263,
0.000271589374668171,0.000352213067600988,0.000388398097499851,0.000404123622054936,
0.000459162957997731,0.000486682625969128,0.000500442459954827,0.000514202293940526),
 .UNSPECIFIED.);
#4315=B_SPLINE_CURVE_WITH_KNOTS('',3,(#170457,#170458,#170459,#170460,#170461,
#170462,#170463,#170464,#170465,#170466,#170467,#170468,#170469,#170470,
#170471,#170472,#170473,#170474,#170475,#170476,#170477,#170478,#170479,
#170480,#170481,#170482,#170483,#170484,#170485,#170486,#170487,#170488,
#170489,#170490,#170491,#170492,#170493,#170494,#170495,#170496,#170497,
#170498,#170499),.UNSPECIFIED.,.F.,.F.,(4,3,3,3,3,3,3,3,3,3,3,3,3,3,4),
(0.,1.1289069806584E-5,7.65259667159113E-5,0.000102837507928536,0.000112544869199276,
0.000130746171581913,0.000194450729921141,0.000226303009090755,0.000242229148675562,
0.000258155288260369,0.000258291104876519,0.000327654633610196,0.000399363990826946,
0.000469709285178442,0.000516310576520737),.UNSPECIFIED.);
#4316=B_SPLINE_CURVE_WITH_KNOTS('',3,(#170507,#170508,#170509,#170510,#170511,
#170512,#170513,#170514,#170515,#170516,#170517,#170518,#170519,#170520,
#170521,#170522,#170523,#170524,#170525,#170526,#170527,#170528,#170529,
#170530,#170531,#170532,#170533,#170534,#170535,#170536,#170537,#170538,
#170539,#170540,#170541,#170542,#170543,#170544,#170545,#170546),
 .UNSPECIFIED.,.F.,.F.,(4,3,3,3,3,3,3,3,3,3,3,3,3,4),(0.,6.84564250954211E-5,
0.000138288406622434,0.000205407478971246,0.000256966021225848,0.000257101146970262,
0.000271589374668172,0.000352213067604716,0.000388398097499863,0.000404123622054945,
0.000459162957997735,0.000486682625969129,0.000500442459954827,0.000514202293940524),
 .UNSPECIFIED.);
#4317=B_SPLINE_CURVE_WITH_KNOTS('',3,(#170550,#170551,#170552,#170553,#170554,
#170555,#170556,#170557,#170558,#170559,#170560,#170561,#170562,#170563,
#170564,#170565,#170566,#170567,#170568,#170569,#170570,#170571,#170572,
#170573,#170574,#170575,#170576,#170577,#170578,#170579,#170580,#170581,
#170582,#170583,#170584,#170585,#170586,#170587,#170588,#170589,#170590,
#170591,#170592),.UNSPECIFIED.,.F.,.F.,(4,3,3,3,3,3,3,3,3,3,3,3,3,3,4),
(0.,1.1289069806583E-5,7.65259667103485E-5,0.000102837507928521,0.000112544869199261,
0.0001307461715819,0.000194450729921134,0.000226303009090751,0.00024222914867556,
0.000258155288260369,0.000258291104876502,0.000327654633618343,0.000399363990843429,
0.000469709285202199,0.000516310576520737),.UNSPECIFIED.);
#4318=B_SPLINE_CURVE_WITH_KNOTS('',3,(#170600,#170601,#170602,#170603,#170604,
#170605,#170606,#170607,#170608,#170609,#170610,#170611,#170612,#170613,
#170614,#170615,#170616,#170617,#170618,#170619,#170620,#170621,#170622,
#170623,#170624,#170625,#170626,#170627,#170628,#170629,#170630,#170631,
#170632,#170633,#170634,#170635,#170636,#170637,#170638,#170639),
 .UNSPECIFIED.,.F.,.F.,(4,3,3,3,3,3,3,3,3,3,3,3,3,4),(0.,6.84564250890799E-5,
0.000138288406609806,0.000205407478953346,0.000256966021225843,0.000257101146970264,
0.00027158937466816,0.000352213067600159,0.000388398097499754,0.00040412362205485,
0.000459162957997689,0.000486682625969108,0.000500442459954818,0.000514202293940527),
 .UNSPECIFIED.);
#4319=B_SPLINE_CURVE_WITH_KNOTS('',3,(#170643,#170644,#170645,#170646,#170647,
#170648,#170649,#170650,#170651,#170652,#170653,#170654,#170655,#170656,
#170657,#170658,#170659,#170660,#170661,#170662,#170663,#170664,#170665,
#170666,#170667,#170668,#170669,#170670,#170671,#170672,#170673,#170674,
#170675,#170676,#170677,#170678,#170679,#170680,#170681,#170682,#170683,
#170684,#170685),.UNSPECIFIED.,.F.,.F.,(4,3,3,3,3,3,3,3,3,3,3,3,3,3,4),
(0.,1.12890698065784E-5,7.65259667110566E-5,0.000102837507928478,0.000112544869199221,
0.000130746171581864,0.000194450729921115,0.00022630300909074,0.000242229148675553,
0.000258155288260366,0.000258291104876503,0.000327654633619958,0.000399363990846323,
0.000469709285205513,0.000516310576520731),.UNSPECIFIED.);
#4320=B_SPLINE_CURVE_WITH_KNOTS('',3,(#170693,#170694,#170695,#170696,#170697,
#170698,#170699,#170700,#170701,#170702,#170703,#170704,#170705,#170706,
#170707,#170708,#170709,#170710,#170711,#170712,#170713,#170714,#170715,
#170716,#170717,#170718,#170719,#170720,#170721,#170722,#170723,#170724,
#170725,#170726,#170727,#170728,#170729,#170730,#170731,#170732),
 .UNSPECIFIED.,.F.,.F.,(4,3,3,3,3,3,3,3,3,3,3,3,3,4),(0.,6.84564250865478E-5,
0.000138288406603928,0.000205407478942991,0.000256966021225854,0.00025710114697026,
0.000271589374668167,0.000352213067606407,0.000388398097499869,0.000404123622054951,
0.000459162957997736,0.000486682625969128,0.000500442459954825,0.000514202293940521),
 .UNSPECIFIED.);
#4321=B_SPLINE_CURVE_WITH_KNOTS('',3,(#170736,#170737,#170738,#170739,#170740,
#170741,#170742,#170743,#170744,#170745,#170746,#170747,#170748,#170749,
#170750,#170751,#170752,#170753,#170754,#170755,#170756,#170757,#170758,
#170759,#170760,#170761,#170762,#170763,#170764,#170765,#170766,#170767,
#170768,#170769,#170770,#170771,#170772,#170773,#170774,#170775,#170776,
#170777,#170778),.UNSPECIFIED.,.F.,.F.,(4,3,3,3,3,3,3,3,3,3,3,3,3,3,4),
(0.,1.12890698065819E-5,7.65259667075592E-5,0.000102837507928482,0.000112544869199225,
0.000130746171581869,0.000194450729921122,0.000226303009090748,0.000242229148675561,
0.000258155288260374,0.000258291104876516,0.000327654633605226,0.000399363990816631,
0.000469709285163391,0.000516310576520749),.UNSPECIFIED.);
#4322=B_SPLINE_CURVE_WITH_KNOTS('',3,(#170786,#170787,#170788,#170789,#170790,
#170791,#170792,#170793,#170794,#170795,#170796,#170797,#170798,#170799,
#170800,#170801,#170802,#170803,#170804,#170805,#170806,#170807,#170808,
#170809,#170810,#170811,#170812,#170813,#170814,#170815,#170816,#170817,
#170818,#170819,#170820,#170821,#170822,#170823,#170824,#170825),
 .UNSPECIFIED.,.F.,.F.,(4,3,3,3,3,3,3,3,3,3,3,3,3,4),(0.,6.84564250871706E-5,
0.000138288406605827,0.000205407478946739,0.000256966021225855,0.000257101146970261,
0.000271589374668165,0.000352213067617463,0.000388398097499751,0.000404123622054848,
0.000459162957997684,0.000486682625969103,0.000500442459954812,0.000514202293940521),
 .UNSPECIFIED.);
#4323=B_SPLINE_CURVE_WITH_KNOTS('',3,(#170829,#170830,#170831,#170832,#170833,
#170834,#170835,#170836,#170837,#170838,#170839,#170840,#170841,#170842,
#170843,#170844,#170845,#170846,#170847,#170848,#170849,#170850,#170851,
#170852,#170853,#170854,#170855,#170856,#170857,#170858,#170859,#170860,
#170861,#170862,#170863,#170864,#170865,#170866,#170867,#170868,#170869,
#170870,#170871),.UNSPECIFIED.,.F.,.F.,(4,3,3,3,3,3,3,3,3,3,3,3,3,3,4),
(0.,1.12890698065823E-5,7.65259667154223E-5,0.000102837507928501,0.000112544869199243,
0.000130746171581885,0.000194450729921131,0.000226303009090754,0.000242229148675565,
0.000258155288260377,0.000258291104876513,0.000327654633611621,0.000399363990829974,
0.000469709285183087,0.000516310576520753),.UNSPECIFIED.);
#4324=B_SPLINE_CURVE_WITH_KNOTS('',3,(#170879,#170880,#170881,#170882,#170883,
#170884,#170885,#170886,#170887,#170888,#170889,#170890,#170891,#170892,
#170893,#170894,#170895,#170896,#170897,#170898,#170899,#170900,#170901,
#170902,#170903,#170904,#170905,#170906,#170907,#170908,#170909,#170910,
#170911,#170912,#170913,#170914,#170915,#170916,#170917,#170918),
 .UNSPECIFIED.,.F.,.F.,(4,3,3,3,3,3,3,3,3,3,3,3,3,4),(0.,6.84564250850767E-5,
0.000138288406600822,0.000205407478937571,0.000256966021225869,0.000257101146970269,
0.00027158937466817,0.000352213067610346,0.000388398097499747,0.000404123622054845,
0.000459162957997688,0.000486682625969109,0.00050044245995482,0.000514202293940531),
 .UNSPECIFIED.);
#4325=B_SPLINE_CURVE_WITH_KNOTS('',3,(#170922,#170923,#170924,#170925,#170926,
#170927,#170928,#170929,#170930,#170931,#170932,#170933,#170934,#170935,
#170936,#170937,#170938,#170939,#170940,#170941,#170942,#170943,#170944,
#170945,#170946,#170947,#170948,#170949,#170950,#170951,#170952,#170953,
#170954,#170955,#170956,#170957,#170958,#170959,#170960,#170961,#170962,
#170963,#170964),.UNSPECIFIED.,.F.,.F.,(4,3,3,3,3,3,3,3,3,3,3,3,3,3,4),
(0.,1.12890698065787E-5,7.65259667143295E-5,0.00010283750792846,0.000112544869199205,
0.000130746171581851,0.000194450729921113,0.000226303009090744,0.000242229148675559,
0.000258155288260375,0.00025829110487651,0.000327654633621617,0.000399363990849291,
0.000469709285208686,0.00051631057652075),.UNSPECIFIED.);
#4326=B_SPLINE_CURVE_WITH_KNOTS('',3,(#170972,#170973,#170974,#170975,#170976,
#170977,#170978,#170979,#170980,#170981,#170982,#170983,#170984,#170985,
#170986,#170987,#170988,#170989,#170990,#170991,#170992,#170993,#170994,
#170995,#170996,#170997,#170998,#170999,#171000,#171001,#171002,#171003,
#171004,#171005,#171006,#171007,#171008,#171009,#171010,#171011),
 .UNSPECIFIED.,.F.,.F.,(4,3,3,3,3,3,3,3,3,3,3,3,3,4),(0.,6.84564250915387E-5,
0.00013828840661381,0.000205407478957333,0.00025696602122584,0.000257101146970264,
0.000271589374668166,0.000352213067592918,0.000388398097499716,0.000404123622054817,
0.000459162957997673,0.000486682625969101,0.000500442459954815,0.000514202293940529),
 .UNSPECIFIED.);
#4327=B_SPLINE_CURVE_WITH_KNOTS('',3,(#171015,#171016,#171017,#171018,#171019,
#171020,#171021,#171022,#171023,#171024,#171025,#171026,#171027,#171028,
#171029,#171030,#171031,#171032,#171033,#171034,#171035,#171036,#171037,
#171038,#171039,#171040,#171041,#171042,#171043,#171044,#171045,#171046,
#171047,#171048,#171049,#171050,#171051,#171052,#171053,#171054,#171055,
#171056,#171057),.UNSPECIFIED.,.F.,.F.,(4,3,3,3,3,3,3,3,3,3,3,3,3,3,4),
(0.,1.128906980658E-5,7.65259667093686E-5,0.00010283750792849,0.000112544869199233,
0.000130746171581876,0.000194450729921126,0.000226303009090751,0.000242229148675563,
0.000258155288260376,0.000258291104876518,0.00032765463361249,0.000399363990831544,
0.000469709285185222,0.000516310576520752),.UNSPECIFIED.);
#4328=B_SPLINE_CURVE_WITH_KNOTS('',3,(#171065,#171066,#171067,#171068,#171069,
#171070,#171071,#171072,#171073,#171074,#171075,#171076,#171077,#171078,
#171079,#171080,#171081,#171082,#171083,#171084,#171085,#171086,#171087,
#171088,#171089,#171090,#171091,#171092,#171093,#171094,#171095,#171096,
#171097,#171098,#171099,#171100,#171101,#171102,#171103,#171104),
 .UNSPECIFIED.,.F.,.F.,(4,3,3,3,3,3,3,3,3,3,3,3,3,4),(0.,6.84564250730484E-5,
0.000138288406575729,0.000205407478898954,0.000256966021225863,0.000257101146970266,
0.000271589374668165,0.000352213067626712,0.000388398097499794,0.000404123622054886,
0.000459162957997709,0.00048668262596912,0.000500442459954826,0.000514202293940531),
 .UNSPECIFIED.);
#4329=B_SPLINE_CURVE_WITH_KNOTS('',3,(#171108,#171109,#171110,#171111,#171112,
#171113,#171114,#171115,#171116,#171117,#171118,#171119,#171120,#171121,
#171122,#171123,#171124,#171125,#171126,#171127,#171128,#171129,#171130,
#171131,#171132,#171133,#171134,#171135,#171136,#171137,#171138,#171139,
#171140,#171141,#171142,#171143,#171144,#171145,#171146,#171147,#171148,
#171149,#171150),.UNSPECIFIED.,.F.,.F.,(4,3,3,3,3,3,3,3,3,3,3,3,3,3,4),
(0.,1.12890698065735E-5,7.65259666964498E-5,0.000102837507928437,0.000112544869199182,
0.000130746171581831,0.000194450729921099,0.000226303009090734,0.000242229148675551,
0.000258155288260368,0.000258291104876531,0.000327654633628666,0.00039936399086441,
0.000469709285233363,0.000516310576520736),.UNSPECIFIED.);
#4330=B_SPLINE_CURVE_WITH_KNOTS('',3,(#171158,#171159,#171160,#171161,#171162,
#171163,#171164,#171165,#171166,#171167,#171168,#171169,#171170,#171171,
#171172,#171173,#171174,#171175,#171176,#171177,#171178,#171179,#171180,
#171181,#171182,#171183,#171184,#171185,#171186,#171187,#171188,#171189,
#171190,#171191,#171192,#171193,#171194,#171195,#171196,#171197),
 .UNSPECIFIED.,.F.,.F.,(4,3,3,3,3,3,3,3,3,3,3,3,3,4),(0.,6.84564250925084E-5,
0.000138288406615908,0.000205407478960095,0.000256966021225855,0.000257101146970265,
0.000271589374668168,0.000352213067604673,0.000388398097499809,0.000404123622054899,
0.000459162957997714,0.000486682625969122,0.000500442459954826,0.00051420229394053),
 .UNSPECIFIED.);
#4331=B_SPLINE_CURVE_WITH_KNOTS('',3,(#171201,#171202,#171203,#171204,#171205,
#171206,#171207,#171208,#171209,#171210,#171211,#171212,#171213,#171214,
#171215,#171216,#171217,#171218,#171219,#171220,#171221,#171222,#171223,
#171224,#171225,#171226,#171227,#171228,#171229,#171230,#171231,#171232,
#171233,#171234,#171235,#171236,#171237,#171238,#171239,#171240,#171241,
#171242,#171243),.UNSPECIFIED.,.F.,.F.,(4,3,3,3,3,3,3,3,3,3,3,3,3,3,4),
(0.,1.12890698065805E-5,7.65259667133678E-5,0.000102837507928527,0.000112544869199267,
0.000130746171581905,0.000194450729921139,0.000226303009090756,0.000242229148675565,
0.000258155288260373,0.000258291104876516,0.000327654633621551,0.00039936399085004,
0.000469709285212181,0.000516310576520747),.UNSPECIFIED.);
#4332=B_SPLINE_CURVE_WITH_KNOTS('',3,(#171251,#171252,#171253,#171254,#171255,
#171256,#171257,#171258,#171259,#171260,#171261,#171262,#171263,#171264,
#171265,#171266,#171267,#171268,#171269,#171270,#171271,#171272,#171273,
#171274,#171275,#171276,#171277,#171278,#171279,#171280,#171281,#171282,
#171283,#171284,#171285,#171286,#171287,#171288,#171289,#171290),
 .UNSPECIFIED.,.F.,.F.,(4,3,3,3,3,3,3,3,3,3,3,3,3,4),(0.,6.84564250780475E-5,
0.000138288406587184,0.000205407478918763,0.000256966021225858,0.000257101146970266,
0.000271589374668172,0.000352213067616118,0.000388398097499824,0.000404123622054913,
0.000459162957997722,0.000486682625969127,0.000500442459954829,0.000514202293940532),
 .UNSPECIFIED.);
#4333=B_SPLINE_CURVE_WITH_KNOTS('',3,(#171294,#171295,#171296,#171297,#171298,
#171299,#171300,#171301,#171302,#171303,#171304,#171305,#171306,#171307,
#171308,#171309,#171310,#171311,#171312,#171313,#171314,#171315,#171316,
#171317,#171318,#171319,#171320,#171321,#171322,#171323,#171324,#171325,
#171326,#171327,#171328,#171329,#171330,#171331,#171332,#171333,#171334,
#171335,#171336),.UNSPECIFIED.,.F.,.F.,(4,3,3,3,3,3,3,3,3,3,3,3,3,3,4),
(0.,1.12890698065829E-5,7.6525966699166E-5,0.000102837507928514,0.000112544869199255,
0.000130746171581894,0.000194450729921133,0.000226303009090753,0.000242229148675562,
0.000258155288260372,0.00025829110487651,0.0003276546336249,0.000399363990855324,
0.000469709285217151,0.000516310576520744),.UNSPECIFIED.);
#4334=B_SPLINE_CURVE_WITH_KNOTS('',3,(#171344,#171345,#171346,#171347,#171348,
#171349,#171350,#171351,#171352,#171353,#171354,#171355,#171356,#171357,
#171358,#171359,#171360,#171361,#171362,#171363,#171364,#171365,#171366,
#171367,#171368,#171369,#171370,#171371,#171372,#171373,#171374,#171375,
#171376,#171377,#171378,#171379,#171380,#171381,#171382,#171383),
 .UNSPECIFIED.,.F.,.F.,(4,3,3,3,3,3,3,3,3,3,3,3,3,4),(1.34144585567483E-17,
6.84564250925487E-5,0.000138288406616583,0.000205407478962631,0.000256966021225856,
0.000257101146970265,0.000271589374668168,0.00035221306759979,0.000388398097499808,
0.000404123622054899,0.000459162957997714,0.000486682625969122,0.000500442459954826,
0.00051420229394053),.UNSPECIFIED.);
#4335=B_SPLINE_CURVE_WITH_KNOTS('',3,(#171387,#171388,#171389,#171390,#171391,
#171392,#171393,#171394,#171395,#171396,#171397,#171398,#171399,#171400,
#171401,#171402,#171403,#171404,#171405,#171406,#171407,#171408,#171409,
#171410,#171411,#171412,#171413,#171414,#171415,#171416,#171417,#171418,
#171419,#171420,#171421,#171422,#171423,#171424,#171425,#171426,#171427,
#171428,#171429),.UNSPECIFIED.,.F.,.F.,(4,3,3,3,3,3,3,3,3,3,3,3,3,3,4),
(0.,1.12890698065832E-5,7.65259667081792E-5,0.000102837507928538,0.000112544869199278,
0.000130746171581915,0.000194450729921144,0.000226303009090759,0.000242229148675566,
0.000258155288260373,0.000258291104876514,0.000327654633623112,0.000399363990853129,
0.00046970928521632,0.000516310576520746),.UNSPECIFIED.);
#4336=B_SPLINE_CURVE_WITH_KNOTS('',3,(#171437,#171438,#171439,#171440,#171441,
#171442,#171443,#171444,#171445,#171446,#171447,#171448,#171449,#171450,
#171451,#171452,#171453,#171454,#171455,#171456,#171457,#171458,#171459,
#171460,#171461,#171462,#171463,#171464,#171465,#171466,#171467,#171468,
#171469,#171470,#171471,#171472,#171473,#171474,#171475,#171476),
 .UNSPECIFIED.,.F.,.F.,(4,3,3,3,3,3,3,3,3,3,3,3,3,4),(0.,6.84564250775598E-5,
0.000138288406585897,0.000205407478917233,0.000256966021225855,0.000257101146970263,
0.000271589374668167,0.000352213067595873,0.000388398097499834,0.000404123622054921,
0.000459162957997723,0.000486682625969125,0.000500442459954825,0.000514202293940526),
 .UNSPECIFIED.);
#4337=B_SPLINE_CURVE_WITH_KNOTS('',3,(#171480,#171481,#171482,#171483,#171484,
#171485,#171486,#171487,#171488,#171489,#171490,#171491,#171492,#171493,
#171494,#171495,#171496,#171497,#171498,#171499,#171500,#171501,#171502,
#171503,#171504,#171505,#171506,#171507,#171508,#171509,#171510,#171511,
#171512,#171513,#171514,#171515,#171516,#171517,#171518,#171519,#171520,
#171521,#171522),.UNSPECIFIED.,.F.,.F.,(4,3,3,3,3,3,3,3,3,3,3,3,3,3,4),
(0.,1.1289069806584E-5,7.65259667025282E-5,0.000102837507928508,0.00011254486919925,
0.000130746171581889,0.000194450729921128,0.000226303009090748,0.000242229148675557,
0.000258155288260367,0.000258291104876519,0.000327654633616274,0.000399363990838822,
0.000469709285195002,0.000516310576520734),.UNSPECIFIED.);
#4338=B_SPLINE_CURVE_WITH_KNOTS('',3,(#171530,#171531,#171532,#171533,#171534,
#171535,#171536,#171537,#171538,#171539,#171540,#171541,#171542,#171543,
#171544,#171545,#171546,#171547,#171548,#171549,#171550,#171551,#171552,
#171553,#171554,#171555,#171556,#171557,#171558,#171559,#171560,#171561,
#171562,#171563,#171564,#171565,#171566,#171567,#171568,#171569),
 .UNSPECIFIED.,.F.,.F.,(4,3,3,3,3,3,3,3,3,3,3,3,3,4),(0.,6.84564250757926E-5,
0.000138288406582254,0.000205407478911281,0.000256966021225868,0.000257101146970264,
0.00027158937466817,0.000352213067604392,0.000388398097499803,0.000404123622054894,
0.000459162957997711,0.00048668262596912,0.000500442459954824,0.000514202293940529),
 .UNSPECIFIED.);
#4339=B_SPLINE_CURVE_WITH_KNOTS('',3,(#171573,#171574,#171575,#171576,#171577,
#171578,#171579,#171580,#171581,#171582,#171583,#171584,#171585,#171586,
#171587,#171588,#171589,#171590,#171591,#171592,#171593,#171594,#171595,
#171596,#171597,#171598,#171599,#171600,#171601,#171602,#171603,#171604,
#171605,#171606,#171607,#171608,#171609,#171610,#171611,#171612,#171613,
#171614,#171615),.UNSPECIFIED.,.F.,.F.,(4,3,3,3,3,3,3,3,3,3,3,3,3,3,4),
(0.,1.12890698065807E-5,7.65259667028005E-5,0.000102837507928501,0.000112544869199243,
0.000130746171581885,0.00019445072992113,0.000226303009090753,0.000242229148675564,
0.000258155288260375,0.00025829110487652,0.000327654633608315,0.000399363990823035,
0.00046970928517307,0.00051631057652075),.UNSPECIFIED.);
#4340=B_SPLINE_CURVE_WITH_KNOTS('',3,(#171623,#171624,#171625,#171626,#171627,
#171628,#171629,#171630,#171631,#171632,#171633,#171634,#171635,#171636,
#171637,#171638,#171639,#171640,#171641,#171642,#171643,#171644,#171645,
#171646,#171647,#171648,#171649,#171650,#171651,#171652,#171653,#171654,
#171655,#171656,#171657,#171658,#171659,#171660,#171661,#171662),
 .UNSPECIFIED.,.F.,.F.,(4,3,3,3,3,3,3,3,3,3,3,3,3,4),(0.,6.84564250793529E-5,
0.000138288406589974,0.000205407478923682,0.000256966021225855,0.000257101146970264,
0.000271589374668171,0.000352213067612092,0.000388398097499841,0.000404123622054927,
0.000459162957997727,0.000486682625969127,0.000500442459954827,0.000514202293940527),
 .UNSPECIFIED.);
#4341=B_SPLINE_CURVE_WITH_KNOTS('',3,(#171666,#171667,#171668,#171669,#171670,
#171671,#171672,#171673,#171674,#171675,#171676,#171677,#171678,#171679,
#171680,#171681,#171682,#171683,#171684,#171685,#171686,#171687,#171688,
#171689,#171690,#171691,#171692,#171693,#171694,#171695,#171696,#171697,
#171698,#171699,#171700,#171701,#171702,#171703,#171704,#171705,#171706,
#171707,#171708),.UNSPECIFIED.,.F.,.F.,(4,3,3,3,3,3,3,3,3,3,3,3,3,3,4),
(1.73472347597681E-18,1.1289069806582E-5,7.65259666980292E-5,0.000102837507928463,
0.000112544869199207,0.000130746171581853,0.000194450729921112,0.000226303009090742,
0.000242229148675557,0.000258155288260371,0.00025829110487652,0.000327654633617188,
0.000399363990840792,0.00046970928519829,0.000516310576520741),
 .UNSPECIFIED.);
#4342=B_SPLINE_CURVE_WITH_KNOTS('',3,(#171716,#171717,#171718,#171719,#171720,
#171721,#171722,#171723,#171724,#171725,#171726,#171727,#171728,#171729,
#171730,#171731,#171732,#171733,#171734,#171735,#171736,#171737,#171738,
#171739,#171740,#171741,#171742,#171743,#171744,#171745,#171746,#171747,
#171748,#171749,#171750,#171751,#171752,#171753,#171754,#171755),
 .UNSPECIFIED.,.F.,.F.,(4,3,3,3,3,3,3,3,3,3,3,3,3,4),(0.,6.84564250891977E-5,
0.00013828840660983,0.000205407478953017,0.000256966021225848,0.000257101146970265,
0.000271589374668171,0.000352213067589024,0.000388398097499806,0.000404123622054896,
0.000459162957997713,0.000486682625969122,0.000500442459954826,0.000514202293940531),
 .UNSPECIFIED.);
#4343=B_SPLINE_CURVE_WITH_KNOTS('',3,(#171759,#171760,#171761,#171762,#171763,
#171764,#171765,#171766,#171767,#171768,#171769,#171770,#171771,#171772,
#171773,#171774,#171775,#171776,#171777,#171778,#171779,#171780,#171781,
#171782,#171783,#171784,#171785,#171786,#171787,#171788,#171789,#171790,
#171791,#171792,#171793,#171794,#171795,#171796,#171797,#171798,#171799,
#171800,#171801),.UNSPECIFIED.,.F.,.F.,(4,3,3,3,3,3,3,3,3,3,3,3,3,3,4),
(0.,1.12890698065773E-5,7.65259666988184E-5,0.000102837507928458,0.000112544869199202,
0.000130746171581848,0.00019445072992111,0.00022630300909074,0.000242229148675555,
0.000258155288260371,0.00025829110487651,0.000327654633612431,0.000399363990831073,
0.000469709285184065,0.000516310576520741),.UNSPECIFIED.);
#4344=B_SPLINE_CURVE_WITH_KNOTS('',3,(#171808,#171809,#171810,#171811,#171812,
#171813,#171814,#171815,#171816,#171817,#171818,#171819,#171820,#171821,
#171822,#171823,#171824,#171825,#171826,#171827,#171828,#171829,#171830,
#171831,#171832,#171833,#171834,#171835,#171836,#171837,#171838,#171839,
#171840,#171841,#171842,#171843,#171844,#171845,#171846,#171847),
 .UNSPECIFIED.,.F.,.F.,(4,3,3,3,3,3,3,3,3,3,3,3,3,4),(0.,6.84564250836823E-5,
0.000138288406598479,0.00020540747893587,0.000256966021225843,0.000257101146970263,
0.000271589374668168,0.000352213067600198,0.000388398097499801,0.000404123622054892,
0.000459162957997709,0.000486682625969117,0.000500442459954822,0.000514202293940526),
 .UNSPECIFIED.);
#4345=B_SPLINE_CURVE_WITH_KNOTS('',3,(#171849,#171850,#171851,#171852,#171853,
#171854,#171855,#171856,#171857,#171858,#171859,#171860,#171861,#171862,
#171863,#171864,#171865,#171866,#171867,#171868,#171869,#171870,#171871,
#171872,#171873,#171874,#171875,#171876,#171877,#171878,#171879,#171880,
#171881,#171882,#171883,#171884,#171885,#171886,#171887,#171888,#171889,
#171890,#171891),.UNSPECIFIED.,.F.,.F.,(4,3,3,3,3,3,3,3,3,3,3,3,3,3,4),
(0.,1.12890698065822E-5,7.65259667098589E-5,0.000102837507928504,0.000112544869199245,
0.000130746171581886,0.000194450729921127,0.000226303009090747,0.000242229148675558,
0.000258155288260368,0.000258291104876532,0.00032765463361062,0.000399363990827817,
0.00046970928517974,0.000516310576520736),.UNSPECIFIED.);
#4346=B_SPLINE_CURVE_WITH_KNOTS('',3,(#171899,#171900,#171901,#171902,#171903,
#171904,#171905,#171906,#171907,#171908,#171909,#171910,#171911,#171912,
#171913,#171914,#171915,#171916,#171917,#171918,#171919,#171920,#171921,
#171922,#171923,#171924,#171925,#171926,#171927,#171928,#171929,#171930,
#171931,#171932,#171933,#171934,#171935,#171936,#171937,#171938),
 .UNSPECIFIED.,.F.,.F.,(4,3,3,3,3,3,3,3,3,3,3,3,3,4),(1.21218245568944E-17,
6.8456425089051E-5,0.000138288406609231,0.000205407478951254,0.000256966021225852,
0.000257101146970263,0.000271589374668161,0.000352213067605418,0.000388398097499745,
0.000404123622054843,0.000459162957997685,0.000486682625969105,0.000500442459954816,
0.000514202293940526),.UNSPECIFIED.);
#4347=B_SPLINE_CURVE_WITH_KNOTS('',3,(#171942,#171943,#171944,#171945,#171946,
#171947,#171948,#171949,#171950,#171951,#171952,#171953,#171954,#171955,
#171956,#171957,#171958,#171959,#171960,#171961,#171962,#171963,#171964,
#171965,#171966,#171967,#171968,#171969,#171970,#171971,#171972,#171973,
#171974,#171975,#171976,#171977,#171978,#171979,#171980,#171981,#171982,
#171983,#171984),.UNSPECIFIED.,.F.,.F.,(4,3,3,3,3,3,3,3,3,3,3,3,3,3,4),
(0.,1.12890698065851E-5,7.65259667091874E-5,0.000102837507928538,0.000112544869199278,
0.000130746171581915,0.000194450729921143,0.000226303009090758,0.000242229148675565,
0.000258155288260372,0.000258291104876525,0.000327654633618784,0.000399363990844283,
0.000469709285203434,0.000516310576520733),.UNSPECIFIED.);
#4348=B_SPLINE_CURVE_WITH_KNOTS('',3,(#171992,#171993,#171994,#171995,#171996,
#171997,#171998,#171999,#172000,#172001,#172002,#172003,#172004,#172005,
#172006,#172007,#172008,#172009,#172010,#172011,#172012,#172013,#172014,
#172015,#172016,#172017,#172018,#172019,#172020,#172021,#172022,#172023,
#172024,#172025,#172026,#172027,#172028,#172029,#172030,#172031),
 .UNSPECIFIED.,.F.,.F.,(4,3,3,3,3,3,3,3,3,3,3,3,3,4),(0.,6.84564250868887E-5,
0.000138288406605147,0.000205407478945967,0.000256966021225847,0.000257101146970261,
0.000271589374668168,0.000352213067598293,0.000388398097499808,0.000404123622054897,
0.00045916295799771,0.000486682625969116,0.000500442459954819,0.000514202293940523),
 .UNSPECIFIED.);
#4349=B_SPLINE_CURVE_WITH_KNOTS('',3,(#172035,#172036,#172037,#172038,#172039,
#172040,#172041,#172042,#172043,#172044,#172045,#172046,#172047,#172048,
#172049,#172050,#172051,#172052,#172053,#172054,#172055,#172056,#172057,
#172058,#172059,#172060,#172061,#172062,#172063,#172064,#172065,#172066,
#172067,#172068,#172069,#172070,#172071,#172072,#172073,#172074,#172075,
#172076,#172077),.UNSPECIFIED.,.F.,.F.,(4,3,3,3,3,3,3,3,3,3,3,3,3,3,4),
(0.,1.12890698065767E-5,7.65259667144555E-5,0.000102837507928448,0.000112544869199193,
0.000130746171581841,0.000194450729921109,0.000226303009090742,0.000242229148675559,
0.000258155288260376,0.000258291104876509,0.00032765463361531,0.000399363990837435,
0.000469709285193806,0.000516310576520752),.UNSPECIFIED.);
#4350=B_SPLINE_CURVE_WITH_KNOTS('',3,(#172085,#172086,#172087,#172088,#172089,
#172090,#172091,#172092,#172093,#172094,#172095,#172096,#172097,#172098,
#172099,#172100,#172101,#172102,#172103,#172104,#172105,#172106,#172107,
#172108,#172109,#172110,#172111,#172112,#172113,#172114,#172115,#172116,
#172117,#172118,#172119,#172120,#172121,#172122,#172123,#172124),
 .UNSPECIFIED.,.F.,.F.,(4,3,3,3,3,3,3,3,3,3,3,3,3,4),(0.,6.84564250823883E-5,
0.000138288406596485,0.000205407478933699,0.000256966021225852,0.00025710114697026,
0.000271589374668168,0.000352213067613843,0.000388398097499785,0.000404123622054877,
0.000459162957997698,0.000486682625969109,0.000500442459954814,0.000514202293940519),
 .UNSPECIFIED.);
#4351=B_SPLINE_CURVE_WITH_KNOTS('',3,(#172128,#172129,#172130,#172131,#172132,
#172133,#172134,#172135,#172136,#172137,#172138,#172139,#172140,#172141,
#172142,#172143,#172144,#172145,#172146,#172147,#172148,#172149,#172150,
#172151,#172152,#172153,#172154,#172155,#172156,#172157,#172158,#172159,
#172160,#172161,#172162,#172163,#172164,#172165,#172166,#172167,#172168,
#172169,#172170),.UNSPECIFIED.,.F.,.F.,(4,3,3,3,3,3,3,3,3,3,3,3,3,3,4),
(0.,1.12890698065798E-5,7.65259667182735E-5,0.000102837507928502,0.000112544869199243,
0.000130746171581884,0.000194450729921128,0.00022630300909075,0.000242229148675561,
0.000258155288260372,0.000258291104876522,0.0003276546336074,0.000399363990821298,
0.000469709285170205,0.000516310576520743),.UNSPECIFIED.);
#4352=B_SPLINE_CURVE_WITH_KNOTS('',3,(#172178,#172179,#172180,#172181,#172182,
#172183,#172184,#172185,#172186,#172187,#172188,#172189,#172190,#172191,
#172192,#172193,#172194,#172195,#172196,#172197,#172198,#172199,#172200,
#172201,#172202,#172203,#172204,#172205,#172206,#172207,#172208,#172209,
#172210,#172211,#172212,#172213,#172214,#172215,#172216,#172217),
 .UNSPECIFIED.,.F.,.F.,(4,3,3,3,3,3,3,3,3,3,3,3,3,4),(0.,6.84564250862393E-5,
0.000138288406603796,0.000205407478943121,0.000256966021225849,0.00025710114697026,
0.000271589374668168,0.000352213067629227,0.000388398097499841,0.000404123622054926,
0.000459162957997723,0.000486682625969121,0.00050044245995482,0.000514202293940519),
 .UNSPECIFIED.);
#4353=B_SPLINE_CURVE_WITH_KNOTS('',3,(#172221,#172222,#172223,#172224,#172225,
#172226,#172227,#172228,#172229,#172230,#172231,#172232,#172233,#172234,
#172235,#172236,#172237,#172238,#172239,#172240,#172241,#172242,#172243,
#172244,#172245,#172246,#172247,#172248,#172249,#172250,#172251,#172252,
#172253,#172254,#172255,#172256,#172257,#172258,#172259,#172260,#172261,
#172262,#172263),.UNSPECIFIED.,.F.,.F.,(4,3,3,3,3,3,3,3,3,3,3,3,3,3,4),
(0.,1.12890698065779E-5,7.6525966711966E-5,0.000102837507928451,0.000112544869199195,
0.000130746171581842,0.000194450729921103,0.000226303009090734,0.00024222914867555,
0.000258155288260365,0.000258291104876504,0.000327654633616026,0.000399363990838618,
0.00046970928519519,0.00051631057652073),.UNSPECIFIED.);
#4354=B_SPLINE_CURVE_WITH_KNOTS('',3,(#172271,#172272,#172273,#172274,#172275,
#172276,#172277,#172278,#172279,#172280,#172281,#172282,#172283,#172284,
#172285,#172286,#172287,#172288,#172289,#172290,#172291,#172292,#172293,
#172294,#172295,#172296,#172297,#172298,#172299,#172300,#172301,#172302,
#172303,#172304,#172305,#172306,#172307,#172308,#172309,#172310),
 .UNSPECIFIED.,.F.,.F.,(4,3,3,3,3,3,3,3,3,3,3,3,3,4),(0.,6.84564250799927E-5,
0.000138288406590908,0.00020540747892476,0.000256966021225863,0.000257101146970264,
0.000271589374668162,0.000352213067603696,0.000388398097499727,0.000404123622054826,
0.000459162957997673,0.000486682625969097,0.000500442459954809,0.000514202293940521),
 .UNSPECIFIED.);
#4355=B_SPLINE_CURVE_WITH_KNOTS('',3,(#172314,#172315,#172316,#172317,#172318,
#172319,#172320,#172321,#172322,#172323,#172324,#172325,#172326,#172327,
#172328,#172329,#172330,#172331,#172332,#172333,#172334,#172335,#172336,
#172337,#172338,#172339,#172340,#172341,#172342,#172343,#172344,#172345,
#172346,#172347,#172348,#172349,#172350,#172351,#172352,#172353,#172354,
#172355,#172356),.UNSPECIFIED.,.F.,.F.,(4,3,3,3,3,3,3,3,3,3,3,3,3,3,4),
(0.,1.12890698065862E-5,7.65259667140177E-5,0.000102837507928526,0.000112544869199266,
0.000130746171581904,0.000194450729921138,0.000226303009090755,0.000242229148675563,
0.000258155288260372,0.000258291104876524,0.000327654633607696,0.000399363990821742,
0.000469709285170638,0.000516310576520743),.UNSPECIFIED.);
#4356=B_SPLINE_CURVE_WITH_KNOTS('',3,(#172364,#172365,#172366,#172367,#172368,
#172369,#172370,#172371,#172372,#172373,#172374,#172375,#172376,#172377,
#172378,#172379,#172380,#172381,#172382,#172383,#172384,#172385,#172386,
#172387,#172388,#172389,#172390,#172391,#172392,#172393,#172394,#172395,
#172396,#172397,#172398,#172399,#172400,#172401,#172402,#172403),
 .UNSPECIFIED.,.F.,.F.,(4,3,3,3,3,3,3,3,3,3,3,3,3,4),(0.,6.84564250927535E-5,
0.000138288406617572,0.000205407478965534,0.000256966021225856,0.000257101146970261,
0.000271589374668161,0.000352213067604348,0.000388398097499758,0.000404123622054853,
0.000459162957997688,0.000486682625969105,0.000500442459954814,0.000514202293940522),
 .UNSPECIFIED.);
#4357=B_SPLINE_CURVE_WITH_KNOTS('',3,(#172407,#172408,#172409,#172410,#172411,
#172412,#172413,#172414,#172415,#172416,#172417,#172418,#172419,#172420,
#172421,#172422,#172423,#172424,#172425,#172426,#172427,#172428,#172429,
#172430,#172431,#172432,#172433,#172434,#172435,#172436,#172437,#172438,
#172439,#172440,#172441,#172442,#172443,#172444,#172445,#172446,#172447,
#172448,#172449),.UNSPECIFIED.,.F.,.F.,(4,3,3,3,3,3,3,3,3,3,3,3,3,3,4),
(0.,1.12890698065764E-5,7.65259667099777E-5,0.00010283750792846,0.000112544869199204,
0.00013074617158185,0.000194450729921111,0.000226303009090741,0.000242229148675556,
0.000258155288260372,0.000258291104876515,0.000327654633618559,0.000399363990844535,
0.000469709285205091,0.000516310576520743),.UNSPECIFIED.);
#4358=B_SPLINE_CURVE_WITH_KNOTS('',3,(#172457,#172458,#172459,#172460,#172461,
#172462,#172463,#172464,#172465,#172466,#172467,#172468,#172469,#172470,
#172471,#172472,#172473,#172474,#172475,#172476,#172477,#172478,#172479,
#172480,#172481,#172482,#172483,#172484,#172485,#172486,#172487,#172488,
#172489,#172490,#172491,#172492,#172493,#172494,#172495,#172496),
 .UNSPECIFIED.,.F.,.F.,(4,3,3,3,3,3,3,3,3,3,3,3,3,4),(0.,6.84564250849387E-5,
0.000138288406600687,0.000205407478937706,0.000256966021225849,0.000257101146970271,
0.000271589374668183,0.000352213067620596,0.000388398097499899,0.000404123622054979,
0.00045916295799776,0.000486682625969151,0.000500442459954846,0.000514202293940541),
 .UNSPECIFIED.);
#4359=B_SPLINE_CURVE_WITH_KNOTS('',3,(#172500,#172501,#172502,#172503,#172504,
#172505,#172506,#172507,#172508,#172509,#172510,#172511,#172512,#172513,
#172514,#172515,#172516,#172517,#172518,#172519,#172520,#172521,#172522,
#172523,#172524,#172525,#172526,#172527,#172528,#172529,#172530,#172531,
#172532,#172533,#172534,#172535,#172536,#172537,#172538,#172539,#172540,
#172541,#172542),.UNSPECIFIED.,.F.,.F.,(4,3,3,3,3,3,3,3,3,3,3,3,3,3,4),
(0.,1.12890698065836E-5,7.65259666749699E-5,0.000102837507928543,0.000112544869199282,
0.000130746171581918,0.000194450729921143,0.000226303009090755,0.000242229148675561,
0.000258155288260367,0.000258291104876523,0.000327654633630791,0.000399363990867584,
0.000469709285236347,0.000516310576520735),.UNSPECIFIED.);
#4360=B_SPLINE_CURVE_WITH_KNOTS('',3,(#172550,#172551,#172552,#172553,#172554,
#172555,#172556,#172557,#172558,#172559,#172560,#172561,#172562,#172563,
#172564,#172565,#172566,#172567,#172568,#172569,#172570,#172571,#172572,
#172573,#172574,#172575,#172576,#172577,#172578,#172579,#172580,#172581,
#172582,#172583,#172584,#172585,#172586,#172587,#172588,#172589),
 .UNSPECIFIED.,.F.,.F.,(4,3,3,3,3,3,3,3,3,3,3,3,3,4),(0.,6.84564250792623E-5,
0.000138288406588807,0.000205407478919674,0.000256966021225846,0.000257101146970266,
0.000271589374668166,0.000352213067610283,0.000388398097499773,0.000404123622054868,
0.0004591629579977,0.000486682625969117,0.000500442459954825,0.000514202293940533),
 .UNSPECIFIED.);
#4361=B_SPLINE_CURVE_WITH_KNOTS('',3,(#172593,#172594,#172595,#172596,#172597,
#172598,#172599,#172600,#172601,#172602,#172603,#172604,#172605,#172606,
#172607,#172608,#172609,#172610,#172611,#172612,#172613,#172614,#172615,
#172616,#172617,#172618,#172619,#172620,#172621,#172622,#172623,#172624,
#172625,#172626,#172627,#172628,#172629,#172630,#172631,#172632,#172633,
#172634,#172635),.UNSPECIFIED.,.F.,.F.,(4,3,3,3,3,3,3,3,3,3,3,3,3,3,4),
(0.,1.12890698065765E-5,7.65259667163295E-5,0.000102837507928452,0.000112544869199197,
0.000130746171581844,0.000194450729921109,0.000226303009090742,0.000242229148675558,
0.000258155288260374,0.000258291104876519,0.0003276546336177,0.000399363990841842,
0.000469709285199261,0.000516310576520749),.UNSPECIFIED.);
#4362=B_SPLINE_CURVE_WITH_KNOTS('',3,(#172643,#172644,#172645,#172646,#172647,
#172648,#172649,#172650,#172651,#172652,#172653,#172654,#172655,#172656,
#172657,#172658,#172659,#172660,#172661,#172662,#172663,#172664,#172665,
#172666,#172667,#172668,#172669,#172670,#172671,#172672,#172673,#172674,
#172675,#172676,#172677,#172678,#172679,#172680,#172681,#172682),
 .UNSPECIFIED.,.F.,.F.,(4,3,3,3,3,3,3,3,3,3,3,3,3,4),(0.,6.84564250789114E-5,
0.000138288406589003,0.000205407478922446,0.000256966021225846,0.000257101146970262,
0.000271589374668163,0.000352213067604696,0.000388398097499755,0.000404123622054851,
0.000459162957997687,0.000486682625969105,0.000500442459954814,0.000514202293940523),
 .UNSPECIFIED.);
#4363=B_SPLINE_CURVE_WITH_KNOTS('',3,(#172686,#172687,#172688,#172689,#172690,
#172691,#172692,#172693,#172694,#172695,#172696,#172697,#172698,#172699,
#172700,#172701,#172702,#172703,#172704,#172705,#172706,#172707,#172708,
#172709,#172710,#172711,#172712,#172713,#172714,#172715,#172716,#172717,
#172718,#172719,#172720,#172721,#172722,#172723,#172724,#172725,#172726,
#172727,#172728),.UNSPECIFIED.,.F.,.F.,(4,3,3,3,3,3,3,3,3,3,3,3,3,3,4),
(0.,1.12890698065812E-5,7.65259666864815E-5,0.000102837507928512,0.000112544869199253,
0.000130746171581893,0.000194450729921133,0.000226303009090753,0.000242229148675563,
0.000258155288260373,0.000258291104876499,0.000327654633628822,0.000399363990862394,
0.000469709285225838,0.000516310576520746),.UNSPECIFIED.);
#4364=B_SPLINE_CURVE_WITH_KNOTS('',3,(#172736,#172737,#172738,#172739,#172740,
#172741,#172742,#172743,#172744,#172745,#172746,#172747,#172748,#172749,
#172750,#172751,#172752,#172753,#172754,#172755,#172756,#172757,#172758,
#172759,#172760,#172761,#172762,#172763,#172764,#172765,#172766,#172767,
#172768,#172769,#172770,#172771,#172772,#172773,#172774,#172775),
 .UNSPECIFIED.,.F.,.F.,(4,3,3,3,3,3,3,3,3,3,3,3,3,4),(0.,6.84564250929779E-5,
0.000138288406617422,0.000205407478963844,0.000256966021225864,0.000257101146970267,
0.000271589374668178,0.000352213067597606,0.00038839809749987,0.000404123622054953,
0.000459162957997743,0.000486682625969139,0.000500442459954836,0.000514202293940534),
 .UNSPECIFIED.);
#4365=B_SPLINE_CURVE_WITH_KNOTS('',3,(#172779,#172780,#172781,#172782,#172783,
#172784,#172785,#172786,#172787,#172788,#172789,#172790,#172791,#172792,
#172793,#172794,#172795,#172796,#172797,#172798,#172799,#172800,#172801,
#172802,#172803,#172804,#172805,#172806,#172807,#172808,#172809,#172810,
#172811,#172812,#172813,#172814,#172815,#172816,#172817,#172818,#172819,
#172820,#172821),.UNSPECIFIED.,.F.,.F.,(4,3,3,3,3,3,3,3,3,3,3,3,3,3,4),
(0.,1.12890698065804E-5,7.65259667067788E-5,0.000102837507928517,0.000112544869199258,
0.000130746171581896,0.000194450729921131,0.000226303009090748,0.000242229148675557,
0.000258155288260366,0.000258291104876526,0.00032765463362171,0.000399363990850038,
0.000469709285211668,0.000516310576520732),.UNSPECIFIED.);
#4366=B_SPLINE_CURVE_WITH_KNOTS('',3,(#172829,#172830,#172831,#172832,#172833,
#172834,#172835,#172836,#172837,#172838,#172839,#172840,#172841,#172842,
#172843,#172844,#172845,#172846,#172847,#172848,#172849,#172850,#172851,
#172852,#172853,#172854,#172855,#172856,#172857,#172858,#172859,#172860,
#172861,#172862,#172863,#172864,#172865,#172866,#172867,#172868),
 .UNSPECIFIED.,.F.,.F.,(4,3,3,3,3,3,3,3,3,3,3,3,3,4),(0.,6.84564250773449E-5,
0.000138288406585096,0.000205407478915048,0.000256966021225853,0.000257101146970262,
0.000271589374668166,0.000352213067599712,0.000388398097499801,0.000404123622054891,
0.000459162957997708,0.000486682625969116,0.00050044245995482,0.000514202293940524),
 .UNSPECIFIED.);
#4367=B_SPLINE_CURVE_WITH_KNOTS('',3,(#172872,#172873,#172874,#172875,#172876,
#172877,#172878,#172879,#172880,#172881,#172882,#172883,#172884,#172885,
#172886,#172887,#172888,#172889,#172890,#172891,#172892,#172893,#172894,
#172895,#172896,#172897,#172898,#172899,#172900,#172901,#172902,#172903,
#172904,#172905,#172906,#172907,#172908,#172909,#172910,#172911,#172912,
#172913,#172914),.UNSPECIFIED.,.F.,.F.,(4,3,3,3,3,3,3,3,3,3,3,3,3,3,4),
(0.,1.12890698065801E-5,7.6525966691684E-5,0.000102837507928504,0.000112544869199246,
0.000130746171581886,0.000194450729921128,0.000226303009090748,0.000242229148675559,
0.000258155288260369,0.000258291104876528,0.000327654633632161,0.000399363990871155,
0.000469709285242306,0.000516310576520738),.UNSPECIFIED.);
#4368=B_SPLINE_CURVE_WITH_KNOTS('',3,(#172922,#172923,#172924,#172925,#172926,
#172927,#172928,#172929,#172930,#172931,#172932,#172933,#172934,#172935,
#172936,#172937,#172938,#172939,#172940,#172941,#172942,#172943,#172944,
#172945,#172946,#172947,#172948,#172949,#172950,#172951,#172952,#172953,
#172954,#172955,#172956,#172957,#172958,#172959,#172960,#172961),
 .UNSPECIFIED.,.F.,.F.,(4,3,3,3,3,3,3,3,3,3,3,3,3,4),(0.,6.84564250807333E-5,
0.000138288406592608,0.000205407478927544,0.000256966021225847,0.000257101146970264,
0.000271589374668166,0.000352213067602011,0.000388398097499788,0.000404123622054881,
0.000459162957997704,0.000486682625969116,0.000500442459954822,0.000514202293940528),
 .UNSPECIFIED.);
#4369=B_SPLINE_CURVE_WITH_KNOTS('',3,(#172965,#172966,#172967,#172968,#172969,
#172970,#172971,#172972,#172973,#172974,#172975,#172976,#172977,#172978,
#172979,#172980,#172981,#172982,#172983,#172984,#172985,#172986,#172987,
#172988,#172989,#172990,#172991,#172992,#172993,#172994,#172995,#172996,
#172997,#172998,#172999,#173000,#173001,#173002,#173003,#173004,#173005,
#173006,#173007),.UNSPECIFIED.,.F.,.F.,(4,3,3,3,3,3,3,3,3,3,3,3,3,3,4),
(0.,1.12890698065848E-5,7.65259667016126E-5,0.00010283750792857,0.000112544869199308,
0.000130746171581941,0.000194450729921157,0.000226303009090765,0.000242229148675569,
0.000258155288260373,0.000258291104876515,0.000327654633612286,0.000399363990831393,
0.000469709285185608,0.000516310576520745),.UNSPECIFIED.);
#4370=B_SPLINE_CURVE_WITH_KNOTS('',3,(#173015,#173016,#173017,#173018,#173019,
#173020,#173021,#173022,#173023,#173024,#173025,#173026,#173027,#173028,
#173029,#173030,#173031,#173032,#173033,#173034,#173035,#173036,#173037,
#173038,#173039,#173040,#173041,#173042,#173043,#173044,#173045,#173046,
#173047,#173048,#173049,#173050,#173051,#173052,#173053,#173054),
 .UNSPECIFIED.,.F.,.F.,(4,3,3,3,3,3,3,3,3,3,3,3,3,4),(0.,6.8456425072981E-5,
0.000138288406576581,0.000205407478902633,0.000256966021225849,0.000257101146970262,
0.000271589374668165,0.000352213067615655,0.000388398097499802,0.000404123622054892,
0.000459162957997708,0.000486682625969116,0.00050044245995482,0.000514202293940524),
 .UNSPECIFIED.);
#4371=B_SPLINE_CURVE_WITH_KNOTS('',3,(#173058,#173059,#173060,#173061,#173062,
#173063,#173064,#173065,#173066,#173067,#173068,#173069,#173070,#173071,
#173072,#173073,#173074,#173075,#173076,#173077,#173078,#173079,#173080,
#173081,#173082,#173083,#173084,#173085,#173086,#173087,#173088,#173089,
#173090,#173091,#173092,#173093,#173094,#173095,#173096,#173097,#173098,
#173099,#173100),.UNSPECIFIED.,.F.,.F.,(4,3,3,3,3,3,3,3,3,3,3,3,3,3,4),
(1.73472347597681E-18,1.12890698065816E-5,7.65259667046772E-5,0.000102837507928469,
0.000112544869199213,0.000130746171581857,0.000194450729921112,0.000226303009090739,
0.000242229148675553,0.000258155288260367,0.000258291104876528,0.00032765463361615,
0.000399363990838513,0.000469709285194426,0.000516310576520732),
 .UNSPECIFIED.);
#4372=B_SPLINE_CURVE_WITH_KNOTS('',3,(#173108,#173109,#173110,#173111,#173112,
#173113,#173114,#173115,#173116,#173117,#173118,#173119,#173120,#173121,
#173122,#173123,#173124,#173125,#173126,#173127,#173128,#173129,#173130,
#173131,#173132,#173133,#173134,#173135,#173136,#173137,#173138,#173139,
#173140,#173141,#173142,#173143,#173144,#173145,#173146,#173147),
 .UNSPECIFIED.,.F.,.F.,(4,3,3,3,3,3,3,3,3,3,3,3,3,4),(0.,6.8456425082964E-5,
0.000138288406597018,0.000205407478933636,0.000256966021225847,0.000257101146970261,
0.000271589374668168,0.000352213067601968,0.000388398097499816,0.000404123622054904,
0.000459162957997713,0.000486682625969118,0.00050044245995482,0.000514202293940522),
 .UNSPECIFIED.);
#4373=B_SPLINE_CURVE_WITH_KNOTS('',3,(#173151,#173152,#173153,#173154,#173155,
#173156,#173157,#173158,#173159,#173160,#173161,#173162,#173163,#173164,
#173165,#173166,#173167,#173168,#173169,#173170,#173171,#173172,#173173,
#173174,#173175,#173176,#173177,#173178,#173179,#173180,#173181,#173182,
#173183,#173184,#173185,#173186,#173187,#173188,#173189,#173190,#173191,
#173192,#173193),.UNSPECIFIED.,.F.,.F.,(4,3,3,3,3,3,3,3,3,3,3,3,3,3,4),
(8.67361737988403E-19,1.1289069806576E-5,7.65259667049559E-5,0.00010283750792845,
0.000112544869199195,0.000130746171581841,0.000194450729921104,0.000226303009090735,
0.00024222914867555,0.000258155288260366,0.000258291104876504,0.000327654633611955,
0.000399363990830165,0.000469709285182823,0.000516310576520731),
 .UNSPECIFIED.);
#4374=B_SPLINE_CURVE_WITH_KNOTS('',3,(#173200,#173201,#173202,#173203,#173204,
#173205,#173206,#173207,#173208,#173209,#173210,#173211,#173212,#173213,
#173214,#173215,#173216,#173217,#173218,#173219,#173220,#173221,#173222,
#173223,#173224,#173225,#173226,#173227,#173228,#173229,#173230,#173231,
#173232,#173233,#173234,#173235,#173236,#173237,#173238,#173239),
 .UNSPECIFIED.,.F.,.F.,(4,3,3,3,3,3,3,3,3,3,3,3,3,4),(0.,6.84564250762055E-5,
0.000138288406583219,0.000205407478913333,0.000256966021225853,0.000257101146970262,
0.000271589374668166,0.000352213067595464,0.000388398097499808,0.000404123622054897,
0.00045916295799771,0.000486682625969117,0.00050044245995482,0.000514202293940523),
 .UNSPECIFIED.);
#4375=B_SPLINE_CURVE_WITH_KNOTS('',3,(#173242,#173243,#173244,#173245,#173246,
#173247,#173248,#173249,#173250,#173251,#173252,#173253,#173254,#173255,
#173256,#173257,#173258,#173259,#173260,#173261,#173262,#173263,#173264,
#173265,#173266,#173267,#173268,#173269,#173270,#173271,#173272,#173273,
#173274,#173275,#173276,#173277,#173278),.UNSPECIFIED.,.F.,.F.,(4,3,3,3,
3,3,3,3,3,3,3,3,4),(0.,1.12535551670963E-5,7.76936938449189E-5,0.000102513517961119,
0.000121879189824267,0.000189659041345284,0.000223548967105793,0.000257294099096092,
0.000257438892866302,0.000325720851757748,0.00039648677396,0.000466242707669274,
0.000514877785732603),.UNSPECIFIED.);
#4376=B_SPLINE_CURVE_WITH_KNOTS('',3,(#173286,#173287,#173288,#173289,#173290,
#173291,#173292,#173293,#173294,#173295,#173296,#173297,#173298,#173299,
#173300,#173301,#173302,#173303,#173304,#173305,#173306,#173307,#173308,
#173309,#173310,#173311,#173312,#173313,#173314,#173315,#173316,#173317,
#173318,#173319,#173320,#173321,#173322,#173323,#173324,#173325),
 .UNSPECIFIED.,.F.,.F.,(4,3,3,3,3,3,3,3,3,3,3,3,3,4),(0.,6.80370855381457E-5,
0.000137303169301757,0.00020363670666859,0.000256396220959708,0.000256540237295746,
0.000285209320207747,0.000342105100635664,0.000384776935956602,0.000400778874201954,
0.000456785658060685,0.000484789049990051,0.000498790745954733,0.000512792441919416),
 .UNSPECIFIED.);
#4377=B_SPLINE_CURVE_WITH_KNOTS('',3,(#173329,#173330,#173331,#173332,#173333,
#173334,#173335,#173336,#173337,#173338,#173339,#173340,#173341,#173342,
#173343,#173344,#173345,#173346,#173347,#173348,#173349,#173350,#173351,
#173352,#173353,#173354,#173355,#173356,#173357,#173358,#173359,#173360,
#173361,#173362,#173363,#173364,#173365),.UNSPECIFIED.,.F.,.F.,(4,3,3,3,
3,3,3,3,3,3,3,3,4),(0.,1.12535551670971E-5,7.76936938477942E-5,0.000102513517961123,
0.00012187918982427,0.000189659041345285,0.000223548967105792,0.000257294099096091,
0.000257438892866299,0.000325720851759598,0.000396486773963869,0.000466242707675107,
0.000514877785732599),.UNSPECIFIED.);
#4378=B_SPLINE_CURVE_WITH_KNOTS('',3,(#173373,#173374,#173375,#173376,#173377,
#173378,#173379,#173380,#173381,#173382,#173383,#173384,#173385,#173386,
#173387,#173388,#173389,#173390,#173391,#173392,#173393,#173394,#173395,
#173396,#173397,#173398,#173399,#173400,#173401,#173402,#173403,#173404,
#173405,#173406,#173407,#173408,#173409,#173410,#173411,#173412),
 .UNSPECIFIED.,.F.,.F.,(4,3,3,3,3,3,3,3,3,3,3,3,3,4),(0.,6.80370855340055E-5,
0.000137303169293596,0.000203636706656825,0.000256396220959708,0.000256540237295739,
0.000285209320207743,0.000342105100635661,0.0003847769359566,0.000400778874201951,
0.000456785658060683,0.000484789049990049,0.000498790745954732,0.000512792441919415),
 .UNSPECIFIED.);
#4379=B_SPLINE_CURVE_WITH_KNOTS('',3,(#173416,#173417,#173418,#173419,#173420,
#173421,#173422,#173423,#173424,#173425,#173426,#173427,#173428,#173429,
#173430,#173431,#173432,#173433,#173434,#173435,#173436,#173437,#173438,
#173439,#173440,#173441,#173442,#173443,#173444,#173445,#173446,#173447,
#173448,#173449,#173450,#173451,#173452),.UNSPECIFIED.,.F.,.F.,(4,3,3,3,
3,3,3,3,3,3,3,3,4),(0.,1.12535551671009E-5,7.76936938396507E-5,0.000102513517961129,
0.000121879189824276,0.000189659041345289,0.000223548967105796,0.000257294099096101,
0.000257438892866303,0.000325720851765454,0.000396486773975544,0.000466242707691564,
0.000514877785732606),.UNSPECIFIED.);
#4380=B_SPLINE_CURVE_WITH_KNOTS('',3,(#173460,#173461,#173462,#173463,#173464,
#173465,#173466,#173467,#173468,#173469,#173470,#173471,#173472,#173473,
#173474,#173475,#173476,#173477,#173478,#173479,#173480,#173481,#173482,
#173483,#173484,#173485,#173486,#173487,#173488,#173489,#173490,#173491,
#173492,#173493,#173494,#173495,#173496,#173497,#173498,#173499),
 .UNSPECIFIED.,.F.,.F.,(4,3,3,3,3,3,3,3,3,3,3,3,3,4),(0.,6.80370855356198E-5,
0.000137303169296276,0.000203636706659361,0.000256396220959709,0.000256540237295742,
0.000285209320207737,0.000342105100635657,0.000384776935956597,0.00040077887420195,
0.000456785658060683,0.00048478904999005,0.000498790745954734,0.000512792441919417),
 .UNSPECIFIED.);
#4381=B_SPLINE_CURVE_WITH_KNOTS('',3,(#173503,#173504,#173505,#173506,#173507,
#173508,#173509,#173510,#173511,#173512,#173513,#173514,#173515,#173516,
#173517,#173518,#173519,#173520,#173521,#173522,#173523,#173524,#173525,
#173526,#173527,#173528,#173529,#173530,#173531,#173532,#173533,#173534,
#173535,#173536,#173537,#173538,#173539),.UNSPECIFIED.,.F.,.F.,(4,3,3,3,
3,3,3,3,3,3,3,3,4),(0.,1.12535551670961E-5,7.76936938360982E-5,0.000102513517961078,
0.000121879189824231,0.000189659041345266,0.000223548967105784,0.000257294099096098,
0.000257438892866302,0.000325720851762349,0.000396486773968905,0.000466242707681605,
0.000514877785732604),.UNSPECIFIED.);
#4382=B_SPLINE_CURVE_WITH_KNOTS('',3,(#173547,#173548,#173549,#173550,#173551,
#173552,#173553,#173554,#173555,#173556,#173557,#173558,#173559,#173560,
#173561,#173562,#173563,#173564,#173565,#173566,#173567,#173568,#173569,
#173570,#173571,#173572,#173573,#173574,#173575,#173576,#173577,#173578,
#173579,#173580,#173581,#173582,#173583,#173584,#173585,#173586),
 .UNSPECIFIED.,.F.,.F.,(4,3,3,3,3,3,3,3,3,3,3,3,3,4),(0.,6.80370855416975E-5,
0.000137303169308508,0.00020363670667723,0.000256396220959707,0.000256540237295748,
0.000285209320207735,0.000342105100635654,0.000384776935956594,0.000400778874201947,
0.00045678565806068,0.000484789049990047,0.000498790745954731,0.000512792441919414),
 .UNSPECIFIED.);
#4383=B_SPLINE_CURVE_WITH_KNOTS('',3,(#173590,#173591,#173592,#173593,#173594,
#173595,#173596,#173597,#173598,#173599,#173600,#173601,#173602,#173603,
#173604,#173605,#173606,#173607,#173608,#173609,#173610,#173611,#173612,
#173613,#173614,#173615,#173616,#173617,#173618,#173619,#173620,#173621,
#173622,#173623,#173624,#173625,#173626),.UNSPECIFIED.,.F.,.F.,(4,3,3,3,
3,3,3,3,3,3,3,3,4),(0.,1.12535551670951E-5,7.76936938499772E-5,0.000102513517961046,
0.000121879189824203,0.000189659041345254,0.000223548967105779,0.000257294099096101,
0.000257438892866304,0.000325720851757687,0.000396486773959997,0.000466242707669562,
0.000514877785732608),.UNSPECIFIED.);
#4384=B_SPLINE_CURVE_WITH_KNOTS('',3,(#173634,#173635,#173636,#173637,#173638,
#173639,#173640,#173641,#173642,#173643,#173644,#173645,#173646,#173647,
#173648,#173649,#173650,#173651,#173652,#173653,#173654,#173655,#173656,
#173657,#173658,#173659,#173660,#173661,#173662,#173663,#173664,#173665,
#173666,#173667,#173668,#173669,#173670,#173671,#173672,#173673),
 .UNSPECIFIED.,.F.,.F.,(4,3,3,3,3,3,3,3,3,3,3,3,3,4),(0.,6.80370855321537E-5,
0.000137303169289407,0.000203636706649685,0.000256396220959712,0.000256540237295725,
0.000285209320207737,0.000342105100635658,0.0003847769359566,0.000400778874201953,
0.000456785658060688,0.000484789049990056,0.000498790745954739,0.000512792441919423),
 .UNSPECIFIED.);
#4385=B_SPLINE_CURVE_WITH_KNOTS('',3,(#173677,#173678,#173679,#173680,#173681,
#173682,#173683,#173684,#173685,#173686,#173687,#173688,#173689,#173690,
#173691,#173692,#173693,#173694,#173695,#173696,#173697,#173698,#173699,
#173700,#173701,#173702,#173703,#173704,#173705,#173706,#173707,#173708,
#173709,#173710,#173711,#173712,#173713),.UNSPECIFIED.,.F.,.F.,(4,3,3,3,
3,3,3,3,3,3,3,3,4),(0.,1.12535551670998E-5,7.76936938510011E-5,0.000102513517961135,
0.000121879189824282,0.000189659041345296,0.000223548967105803,0.000257294099096103,
0.00025743889286631,0.000325720851757794,0.000396486773960278,0.000466242707669978,
0.000514877785732619),.UNSPECIFIED.);
#4386=B_SPLINE_CURVE_WITH_KNOTS('',3,(#173721,#173722,#173723,#173724,#173725,
#173726,#173727,#173728,#173729,#173730,#173731,#173732,#173733,#173734,
#173735,#173736,#173737,#173738,#173739,#173740,#173741,#173742,#173743,
#173744,#173745,#173746,#173747,#173748,#173749,#173750,#173751,#173752,
#173753,#173754,#173755,#173756,#173757,#173758,#173759,#173760),
 .UNSPECIFIED.,.F.,.F.,(4,3,3,3,3,3,3,3,3,3,3,3,3,4),(0.,6.80370855402335E-5,
0.000137303169306136,0.000203636706675648,0.000256396220959704,0.000256540237295737,
0.000285209320207747,0.000342105100635662,0.000384776935956598,0.000400778874201949,
0.000456785658060679,0.000484789049990043,0.000498790745954725,0.000512792441919408),
 .UNSPECIFIED.);
#4387=B_SPLINE_CURVE_WITH_KNOTS('',3,(#173764,#173765,#173766,#173767,#173768,
#173769,#173770,#173771,#173772,#173773,#173774,#173775,#173776,#173777,
#173778,#173779,#173780,#173781,#173782,#173783,#173784,#173785,#173786,
#173787,#173788,#173789,#173790,#173791,#173792,#173793,#173794,#173795,
#173796,#173797,#173798,#173799,#173800),.UNSPECIFIED.,.F.,.F.,(4,3,3,3,
3,3,3,3,3,3,3,3,4),(0.,1.12535551670965E-5,7.76936938370593E-5,0.00010251351796113,
0.000121879189824277,0.000189659041345291,0.000223548967105798,0.000257294099096113,
0.000257438892866305,0.000325720851760076,0.000396486773964988,0.000466242707677394,
0.000514877785732611),.UNSPECIFIED.);
#4388=B_SPLINE_CURVE_WITH_KNOTS('',3,(#173808,#173809,#173810,#173811,#173812,
#173813,#173814,#173815,#173816,#173817,#173818,#173819,#173820,#173821,
#173822,#173823,#173824,#173825,#173826,#173827,#173828,#173829,#173830,
#173831,#173832,#173833,#173834,#173835,#173836,#173837,#173838,#173839,
#173840,#173841,#173842,#173843,#173844,#173845,#173846,#173847),
 .UNSPECIFIED.,.F.,.F.,(4,3,3,3,3,3,3,3,3,3,3,3,3,4),(0.,6.80370855329636E-5,
0.000137303169291043,0.000203636706652177,0.000256396220959708,0.000256540237295739,
0.000285209320207743,0.000342105100635661,0.0003847769359566,0.000400778874201952,
0.000456785658060685,0.000484789049990051,0.000498790745954734,0.000512792441919417),
 .UNSPECIFIED.);
#4389=B_SPLINE_CURVE_WITH_KNOTS('',3,(#173851,#173852,#173853,#173854,#173855,
#173856,#173857,#173858,#173859,#173860,#173861,#173862,#173863,#173864,
#173865,#173866,#173867,#173868,#173869,#173870,#173871,#173872,#173873,
#173874,#173875,#173876,#173877,#173878,#173879,#173880,#173881,#173882,
#173883,#173884,#173885,#173886,#173887),.UNSPECIFIED.,.F.,.F.,(4,3,3,3,
3,3,3,3,3,3,3,3,4),(0.,1.1253555167096E-5,7.7693693832872E-5,0.000102513517961065,
0.000121879189824221,0.000189659041345265,0.000223548967105787,0.000257294099096107,
0.000257438892866309,0.000325720851759186,0.000396486773962424,0.000466242707672148,
0.000514877785732618),.UNSPECIFIED.);
#4390=B_SPLINE_CURVE_WITH_KNOTS('',3,(#173895,#173896,#173897,#173898,#173899,
#173900,#173901,#173902,#173903,#173904,#173905,#173906,#173907,#173908,
#173909,#173910,#173911,#173912,#173913,#173914,#173915,#173916,#173917,
#173918,#173919,#173920,#173921,#173922,#173923,#173924,#173925,#173926,
#173927,#173928,#173929,#173930,#173931,#173932,#173933,#173934),
 .UNSPECIFIED.,.F.,.F.,(4,3,3,3,3,3,3,3,3,3,3,3,3,4),(0.,6.80370855426867E-5,
0.000137303169311313,0.000203636706683517,0.000256396220959705,0.00025654023729572,
0.000285209320207733,0.000342105100635652,0.000384776935956592,0.000400778874201944,
0.000456785658060677,0.000484789049990044,0.000498790745954727,0.00051279244191941),
 .UNSPECIFIED.);
#4391=B_SPLINE_CURVE_WITH_KNOTS('',3,(#173938,#173939,#173940,#173941,#173942,
#173943,#173944,#173945,#173946,#173947,#173948,#173949,#173950,#173951,
#173952,#173953,#173954,#173955,#173956,#173957,#173958,#173959,#173960,
#173961,#173962,#173963,#173964,#173965,#173966,#173967,#173968,#173969,
#173970,#173971,#173972,#173973,#173974),.UNSPECIFIED.,.F.,.F.,(4,3,3,3,
3,3,3,3,3,3,3,3,4),(0.,1.12535551670979E-5,7.76936938511101E-5,0.000102513517961128,
0.000121879189824275,0.000189659041345292,0.0002235489671058,0.000257294099096117,
0.000257438892866308,0.000325720851744255,0.000396486773933114,0.000466242707631399,
0.000514877785732617),.UNSPECIFIED.);
#4392=B_SPLINE_CURVE_WITH_KNOTS('',3,(#173982,#173983,#173984,#173985,#173986,
#173987,#173988,#173989,#173990,#173991,#173992,#173993,#173994,#173995,
#173996,#173997,#173998,#173999,#174000,#174001,#174002,#174003,#174004,
#174005,#174006,#174007,#174008,#174009,#174010,#174011,#174012,#174013,
#174014,#174015,#174016,#174017,#174018,#174019,#174020,#174021),
 .UNSPECIFIED.,.F.,.F.,(4,3,3,3,3,3,3,3,3,3,3,3,3,4),(0.,6.80370855405851E-5,
0.000137303169307101,0.000203636706677472,0.000256396220959704,0.00025654023729574,
0.000285209320207737,0.000342105100635655,0.000384776935956593,0.000400778874201945,
0.000456785658060677,0.000484789049990043,0.000498790745954726,0.000512792441919409),
 .UNSPECIFIED.);
#4393=B_SPLINE_CURVE_WITH_KNOTS('',3,(#174025,#174026,#174027,#174028,#174029,
#174030,#174031,#174032,#174033,#174034,#174035,#174036,#174037,#174038,
#174039,#174040,#174041,#174042,#174043,#174044,#174045,#174046,#174047,
#174048,#174049,#174050,#174051,#174052,#174053,#174054,#174055,#174056,
#174057,#174058,#174059,#174060,#174061),.UNSPECIFIED.,.F.,.F.,(4,3,3,3,
3,3,3,3,3,3,3,3,4),(0.,1.12535551670968E-5,7.76936938519756E-5,0.000102513517961092,
0.000121879189824243,0.000189659041345274,0.00022354896710579,0.000257294099096106,
0.000257438892866305,0.000325720851759131,0.000396486773963648,0.000466242707676064,
0.000514877785732611),.UNSPECIFIED.);
#4394=B_SPLINE_CURVE_WITH_KNOTS('',3,(#174069,#174070,#174071,#174072,#174073,
#174074,#174075,#174076,#174077,#174078,#174079,#174080,#174081,#174082,
#174083,#174084,#174085,#174086,#174087,#174088,#174089,#174090,#174091,
#174092,#174093,#174094,#174095,#174096,#174097,#174098,#174099,#174100,
#174101,#174102,#174103,#174104,#174105,#174106,#174107,#174108),
 .UNSPECIFIED.,.F.,.F.,(4,3,3,3,3,3,3,3,3,3,3,3,3,4),(0.,6.80370855443293E-5,
0.000137303169314145,0.000203636706686637,0.000256396220959703,0.000256540237295738,
0.000285209320207752,0.000342105100635665,0.0003847769359566,0.000400778874201951,
0.000456785658060678,0.000484789049990041,0.000498790745954723,0.000512792441919405),
 .UNSPECIFIED.);
#4395=B_SPLINE_CURVE_WITH_KNOTS('',3,(#174112,#174113,#174114,#174115,#174116,
#174117,#174118,#174119,#174120,#174121,#174122,#174123,#174124,#174125,
#174126,#174127,#174128,#174129,#174130,#174131,#174132,#174133,#174134,
#174135,#174136,#174137,#174138,#174139,#174140,#174141,#174142,#174143,
#174144,#174145,#174146,#174147,#174148),.UNSPECIFIED.,.F.,.F.,(4,3,3,3,
3,3,3,3,3,3,3,3,4),(0.,1.12535551670953E-5,7.76936938441846E-5,0.000102513517961061,
0.000121879189824217,0.000189659041345262,0.000223548967105784,0.000257294099096109,
0.000257438892866307,0.000325720851756007,0.000396486773956202,0.000466242707663296,
0.000514877785732614),.UNSPECIFIED.);
#4396=B_SPLINE_CURVE_WITH_KNOTS('',3,(#174156,#174157,#174158,#174159,#174160,
#174161,#174162,#174163,#174164,#174165,#174166,#174167,#174168,#174169,
#174170,#174171,#174172,#174173,#174174,#174175,#174176,#174177,#174178,
#174179,#174180,#174181,#174182,#174183,#174184,#174185,#174186,#174187,
#174188,#174189,#174190,#174191,#174192,#174193,#174194,#174195),
 .UNSPECIFIED.,.F.,.F.,(4,3,3,3,3,3,3,3,3,3,3,3,3,4),(0.,6.80370855340898E-5,
0.00013730316929358,0.000203636706656239,0.000256396220959703,0.000256540237295742,
0.000285209320207727,0.000342105100635647,0.000384776935956586,0.000400778874201939,
0.000456785658060672,0.000484789049990039,0.000498790745954723,0.000512792441919406),
 .UNSPECIFIED.);
#4397=B_SPLINE_CURVE_WITH_KNOTS('',3,(#174199,#174200,#174201,#174202,#174203,
#174204,#174205,#174206,#174207,#174208,#174209,#174210,#174211,#174212,
#174213,#174214,#174215,#174216,#174217,#174218,#174219,#174220,#174221,
#174222,#174223,#174224,#174225,#174226,#174227,#174228,#174229,#174230,
#174231,#174232,#174233,#174234,#174235),.UNSPECIFIED.,.F.,.F.,(4,3,3,3,
3,3,3,3,3,3,3,3,4),(0.,1.12535551670914E-5,7.76936938407497E-5,0.000102513517961058,
0.000121879189824214,0.000189659041345258,0.00022354896710578,0.000257294099096095,
0.000257438892866303,0.000325720851759145,0.00039648677396219,0.000466242707671321,
0.000514877785732594),.UNSPECIFIED.);
#4398=B_SPLINE_CURVE_WITH_KNOTS('',3,(#174243,#174244,#174245,#174246,#174247,
#174248,#174249,#174250,#174251,#174252,#174253,#174254,#174255,#174256,
#174257,#174258,#174259,#174260,#174261,#174262,#174263,#174264,#174265,
#174266,#174267,#174268,#174269,#174270,#174271,#174272,#174273,#174274,
#174275,#174276,#174277,#174278,#174279,#174280,#174281,#174282),
 .UNSPECIFIED.,.F.,.F.,(4,3,3,3,3,3,3,3,3,3,3,3,3,4),(0.,6.80370855425274E-5,
0.000137303169310403,0.000203636706680631,0.000256396220959705,0.000256540237295745,
0.000285209320207746,0.000342105100635662,0.000384776935956599,0.000400778874201951,
0.000456785658060681,0.000484789049990046,0.000498790745954728,0.000512792441919411),
 .UNSPECIFIED.);
#4399=B_SPLINE_CURVE_WITH_KNOTS('',3,(#174286,#174287,#174288,#174289,#174290,
#174291,#174292,#174293,#174294,#174295,#174296,#174297,#174298,#174299,
#174300,#174301,#174302,#174303,#174304,#174305,#174306,#174307,#174308,
#174309,#174310,#174311,#174312,#174313,#174314,#174315,#174316,#174317,
#174318,#174319,#174320,#174321,#174322),.UNSPECIFIED.,.F.,.F.,(4,3,3,3,
3,3,3,3,3,3,3,3,4),(0.,1.12535551670943E-5,7.76936938459712E-5,0.000102513517961047,
0.000121879189824205,0.000189659041345256,0.000223548967105781,0.000257294099096093,
0.000257438892866307,0.000325720851750959,0.000396486773946435,0.000466242707650226,
0.000514877785732613),.UNSPECIFIED.);
#4400=B_SPLINE_CURVE_WITH_KNOTS('',3,(#174330,#174331,#174332,#174333,#174334,
#174335,#174336,#174337,#174338,#174339,#174340,#174341,#174342,#174343,
#174344,#174345,#174346,#174347,#174348,#174349,#174350,#174351,#174352,
#174353,#174354,#174355,#174356,#174357,#174358,#174359,#174360,#174361,
#174362,#174363,#174364,#174365,#174366,#174367,#174368,#174369),
 .UNSPECIFIED.,.F.,.F.,(4,3,3,3,3,3,3,3,3,3,3,3,3,4),(0.,6.80370855416932E-5,
0.000137303169308873,0.000203636706679008,0.000256396220959704,0.000256540237295732,
0.000285209320207732,0.000342105100635651,0.00038477693595659,0.000400778874201943,
0.000456785658060676,0.000484789049990042,0.000498790745954725,0.000512792441919408),
 .UNSPECIFIED.);
#4401=B_SPLINE_CURVE_WITH_KNOTS('',3,(#174373,#174374,#174375,#174376,#174377,
#174378,#174379,#174380,#174381,#174382,#174383,#174384,#174385,#174386,
#174387,#174388,#174389,#174390,#174391,#174392,#174393,#174394,#174395,
#174396,#174397,#174398,#174399,#174400,#174401,#174402,#174403,#174404,
#174405,#174406,#174407,#174408,#174409),.UNSPECIFIED.,.F.,.F.,(4,3,3,3,
3,3,3,3,3,3,3,3,4),(0.,1.12535551670975E-5,7.76936938474744E-5,0.000102513517961061,
0.000121879189824216,0.000189659041345261,0.000223548967105783,0.000257294099096097,
0.000257438892866305,0.00032572085175803,0.000396486773960401,0.000466242707669455,
0.00051487778573261),.UNSPECIFIED.);
#4402=B_SPLINE_CURVE_WITH_KNOTS('',3,(#174417,#174418,#174419,#174420,#174421,
#174422,#174423,#174424,#174425,#174426,#174427,#174428,#174429,#174430,
#174431,#174432,#174433,#174434,#174435,#174436,#174437,#174438,#174439,
#174440,#174441,#174442,#174443,#174444,#174445,#174446,#174447,#174448,
#174449,#174450,#174451,#174452,#174453,#174454,#174455,#174456),
 .UNSPECIFIED.,.F.,.F.,(4,3,3,3,3,3,3,3,3,3,3,3,3,4),(0.,6.80370855424907E-5,
0.0001373031693105,0.000203636706681343,0.000256396220959704,0.000256540237295739,
0.000285209320207733,0.000342105100635651,0.000384776935956591,0.000400778874201943,
0.000456785658060675,0.000484789049990042,0.000498790745954725,0.000512792441919408),
 .UNSPECIFIED.);
#4403=B_SPLINE_CURVE_WITH_KNOTS('',3,(#174460,#174461,#174462,#174463,#174464,
#174465,#174466,#174467,#174468,#174469,#174470,#174471,#174472,#174473,
#174474,#174475,#174476,#174477,#174478,#174479,#174480,#174481,#174482,
#174483,#174484,#174485,#174486,#174487,#174488,#174489,#174490,#174491,
#174492,#174493,#174494,#174495,#174496),.UNSPECIFIED.,.F.,.F.,(4,3,3,3,
3,3,3,3,3,3,3,3,4),(0.,1.12535551670997E-5,7.76936938476196E-5,0.000102513517961137,
0.000121879189824283,0.000189659041345294,0.0002235489671058,0.000257294099096102,
0.000257438892866305,0.000325720851755202,0.000396486773954731,0.000466242707661486,
0.000514877785732611),.UNSPECIFIED.);
#4404=B_SPLINE_CURVE_WITH_KNOTS('',3,(#174504,#174505,#174506,#174507,#174508,
#174509,#174510,#174511,#174512,#174513,#174514,#174515,#174516,#174517,
#174518,#174519,#174520,#174521,#174522,#174523,#174524,#174525,#174526,
#174527,#174528,#174529,#174530,#174531,#174532,#174533,#174534,#174535,
#174536,#174537,#174538,#174539,#174540,#174541,#174542,#174543),
 .UNSPECIFIED.,.F.,.F.,(4,3,3,3,3,3,3,3,3,3,3,3,3,4),(0.,6.80370855428342E-5,
0.000137303169311103,0.000203636706682138,0.000256396220959707,0.000256540237295733,
0.000285209320207737,0.000342105100635656,0.000384776935956596,0.000400778874201948,
0.000456785658060681,0.000484789049990048,0.000498790745954731,0.000512792441919414),
 .UNSPECIFIED.);
#4405=B_SPLINE_CURVE_WITH_KNOTS('',3,(#174547,#174548,#174549,#174550,#174551,
#174552,#174553,#174554,#174555,#174556,#174557,#174558,#174559,#174560,
#174561,#174562,#174563,#174564,#174565,#174566,#174567,#174568,#174569,
#174570,#174571,#174572,#174573,#174574,#174575,#174576,#174577,#174578,
#174579,#174580,#174581,#174582,#174583),.UNSPECIFIED.,.F.,.F.,(4,3,3,3,
3,3,3,3,3,3,3,3,4),(0.,1.12535551670975E-5,7.7693693847771E-5,0.00010251351796109,
0.000121879189824242,0.000189659041345272,0.000223548967105788,0.000257294099096109,
0.000257438892866303,0.000325720851758554,0.000396486773961584,0.00046624270767156,
0.000514877785732606),.UNSPECIFIED.);
#4406=B_SPLINE_CURVE_WITH_KNOTS('',3,(#174591,#174592,#174593,#174594,#174595,
#174596,#174597,#174598,#174599,#174600,#174601,#174602,#174603,#174604,
#174605,#174606,#174607,#174608,#174609,#174610,#174611,#174612,#174613,
#174614,#174615,#174616,#174617,#174618,#174619,#174620,#174621,#174622,
#174623,#174624,#174625,#174626,#174627,#174628,#174629,#174630),
 .UNSPECIFIED.,.F.,.F.,(4,3,3,3,3,3,3,3,3,3,3,3,3,4),(0.,6.80370855342209E-5,
0.000137303169293638,0.00020363670665596,0.000256396220959704,0.000256540237295741,
0.000285209320207738,0.000342105100635655,0.000384776935956594,0.000400778874201945,
0.000456785658060677,0.000484789049990042,0.000498790745954725,0.000512792441919408),
 .UNSPECIFIED.);
#4407=B_SPLINE_CURVE_WITH_KNOTS('',3,(#174634,#174635,#174636,#174637,#174638,
#174639,#174640,#174641,#174642,#174643,#174644,#174645,#174646,#174647,
#174648,#174649,#174650,#174651,#174652,#174653,#174654,#174655,#174656,
#174657,#174658,#174659,#174660,#174661,#174662,#174663,#174664,#174665,
#174666,#174667,#174668,#174669,#174670),.UNSPECIFIED.,.F.,.F.,(4,3,3,3,
3,3,3,3,3,3,3,3,4),(0.,1.12535551670985E-5,7.76936938451044E-5,0.000102513517961084,
0.000121879189824236,0.000189659041345269,0.000223548967105785,0.000257294099096095,
0.000257438892866301,0.000325720851759207,0.000396486773962963,0.000466242707673494,
0.000514877785732603),.UNSPECIFIED.);
#4408=B_SPLINE_CURVE_WITH_KNOTS('',3,(#174678,#174679,#174680,#174681,#174682,
#174683,#174684,#174685,#174686,#174687,#174688,#174689,#174690,#174691,
#174692,#174693,#174694,#174695,#174696,#174697,#174698,#174699,#174700,
#174701,#174702,#174703,#174704,#174705,#174706,#174707,#174708,#174709,
#174710,#174711,#174712,#174713,#174714,#174715,#174716,#174717),
 .UNSPECIFIED.,.F.,.F.,(4,3,3,3,3,3,3,3,3,3,3,3,3,4),(0.,6.80370855408533E-5,
0.000137303169307367,0.000203636706676852,0.000256396220959703,0.000256540237295735,
0.000285209320207737,0.000342105100635654,0.000384776935956592,0.000400778874201944,
0.000456785658060675,0.000484789049990041,0.000498790745954724,0.000512792441919407),
 .UNSPECIFIED.);
#4409=B_SPLINE_CURVE_WITH_KNOTS('',3,(#174721,#174722,#174723,#174724,#174725,
#174726,#174727,#174728,#174729,#174730,#174731,#174732,#174733,#174734,
#174735,#174736,#174737,#174738,#174739,#174740,#174741,#174742,#174743,
#174744,#174745,#174746,#174747,#174748,#174749,#174750,#174751,#174752,
#174753,#174754,#174755,#174756,#174757),.UNSPECIFIED.,.F.,.F.,(4,3,3,3,
3,3,3,3,3,3,3,3,4),(0.,1.12535551670974E-5,7.76936938464889E-5,0.000102513517961109,
0.000121879189824259,0.000189659041345283,0.000223548967105796,0.00025729409909611,
0.000257438892866308,0.000325720851760378,0.000396486773965212,0.000466242707676601,
0.000514877785732616),.UNSPECIFIED.);
#4410=B_SPLINE_CURVE_WITH_KNOTS('',3,(#174765,#174766,#174767,#174768,#174769,
#174770,#174771,#174772,#174773,#174774,#174775,#174776,#174777,#174778,
#174779,#174780,#174781,#174782,#174783,#174784,#174785,#174786,#174787,
#174788,#174789,#174790,#174791,#174792,#174793,#174794,#174795,#174796,
#174797,#174798,#174799,#174800,#174801,#174802,#174803,#174804),
 .UNSPECIFIED.,.F.,.F.,(4,3,3,3,3,3,3,3,3,3,3,3,3,4),(0.,6.80370855403097E-5,
0.000137303169305359,0.000203636706671983,0.000256396220959709,0.000256540237295736,
0.000285209320207733,0.000342105100635654,0.000384776935956595,0.000400778874201948,
0.000456785658060682,0.00048478904999005,0.000498790745954733,0.000512792441919417),
 .UNSPECIFIED.);
#4411=B_SPLINE_CURVE_WITH_KNOTS('',3,(#174808,#174809,#174810,#174811,#174812,
#174813,#174814,#174815,#174816,#174817,#174818,#174819,#174820,#174821,
#174822,#174823,#174824,#174825,#174826,#174827,#174828,#174829,#174830,
#174831,#174832,#174833,#174834,#174835,#174836,#174837,#174838,#174839,
#174840,#174841,#174842,#174843,#174844),.UNSPECIFIED.,.F.,.F.,(4,3,3,3,
3,3,3,3,3,3,3,3,4),(0.,1.12535551670966E-5,7.76936938395229E-5,0.000102513517961087,
0.00012187918982424,0.000189659041345274,0.00022354896710579,0.00025729409909612,
0.000257438892866307,0.000325720851748994,0.000396486773942172,0.000466242707643575,
0.000514877785732614),.UNSPECIFIED.);
#4412=B_SPLINE_CURVE_WITH_KNOTS('',3,(#174852,#174853,#174854,#174855,#174856,
#174857,#174858,#174859,#174860,#174861,#174862,#174863,#174864,#174865,
#174866,#174867,#174868,#174869,#174870,#174871,#174872,#174873,#174874,
#174875,#174876,#174877,#174878,#174879,#174880,#174881,#174882,#174883,
#174884,#174885,#174886,#174887,#174888,#174889,#174890,#174891),
 .UNSPECIFIED.,.F.,.F.,(4,3,3,3,3,3,3,3,3,3,3,3,3,4),(0.,6.80370855330231E-5,
0.000137303169291361,0.000203636706653042,0.000256396220959707,0.000256540237295735,
0.000285209320207733,0.000342105100635653,0.000384776935956594,0.000400778874201946,
0.00045678565806068,0.000484789049990047,0.00049879074595473,0.000512792441919414),
 .UNSPECIFIED.);
#4413=B_SPLINE_CURVE_WITH_KNOTS('',3,(#174895,#174896,#174897,#174898,#174899,
#174900,#174901,#174902,#174903,#174904,#174905,#174906,#174907,#174908,
#174909,#174910,#174911,#174912,#174913,#174914,#174915,#174916,#174917,
#174918,#174919,#174920,#174921,#174922,#174923,#174924,#174925,#174926,
#174927,#174928,#174929,#174930,#174931),.UNSPECIFIED.,.F.,.F.,(4,3,3,3,
3,3,3,3,3,3,3,3,4),(0.,1.12535551670998E-5,7.76936938476081E-5,0.000102513517961124,
0.000121879189824272,0.000189659041345288,0.000223548967105796,0.000257294099096119,
0.000257438892866305,0.000325720851753445,0.000396486773950165,0.000466242707652896,
0.000514877785732609),.UNSPECIFIED.);
#4414=B_SPLINE_CURVE_WITH_KNOTS('',3,(#174939,#174940,#174941,#174942,#174943,
#174944,#174945,#174946,#174947,#174948,#174949,#174950,#174951,#174952,
#174953,#174954,#174955,#174956,#174957,#174958,#174959,#174960,#174961,
#174962,#174963,#174964,#174965,#174966,#174967,#174968,#174969,#174970,
#174971,#174972,#174973,#174974,#174975,#174976,#174977,#174978),
 .UNSPECIFIED.,.F.,.F.,(4,3,3,3,3,3,3,3,3,3,3,3,3,4),(0.,6.80370855325344E-5,
0.000137303169290103,0.000203636706650601,0.000256396220959707,0.000256540237295731,
0.000285209320207729,0.00034210510063565,0.000384776935956591,0.000400778874201944,
0.000456785658060678,0.000484789049990046,0.00049879074595473,0.000512792441919413),
 .UNSPECIFIED.);
#4415=B_SPLINE_CURVE_WITH_KNOTS('',3,(#174982,#174983,#174984,#174985,#174986,
#174987,#174988,#174989,#174990,#174991,#174992,#174993,#174994,#174995,
#174996,#174997,#174998,#174999,#175000,#175001,#175002,#175003,#175004,
#175005,#175006,#175007,#175008,#175009,#175010,#175011,#175012,#175013,
#175014,#175015,#175016,#175017,#175018),.UNSPECIFIED.,.F.,.F.,(4,3,3,3,
3,3,3,3,3,3,3,3,4),(0.,1.12535551670955E-5,7.76936938495978E-5,0.000102513517961049,
0.000121879189824206,0.000189659041345252,0.000223548967105776,0.000257294099096094,
0.000257438892866299,0.000325720851750144,0.000396486773944257,0.000466242707645802,
0.000514877785732598),.UNSPECIFIED.);
#4416=B_SPLINE_CURVE_WITH_KNOTS('',3,(#175026,#175027,#175028,#175029,#175030,
#175031,#175032,#175033,#175034,#175035,#175036,#175037,#175038,#175039,
#175040,#175041,#175042,#175043,#175044,#175045,#175046,#175047,#175048,
#175049,#175050,#175051,#175052,#175053,#175054,#175055,#175056,#175057,
#175058,#175059,#175060,#175061,#175062,#175063,#175064,#175065),
 .UNSPECIFIED.,.F.,.F.,(4,3,3,3,3,3,3,3,3,3,3,3,3,4),(0.,6.80370855436682E-5,
0.000137303169312912,0.00020363670668485,0.00025639622095971,0.000256540237295729,
0.000285209320207753,0.00034210510063567,0.000384776935956608,0.000400778874201959,
0.00045678565806069,0.000484789049990056,0.000498790745954738,0.000512792441919421),
 .UNSPECIFIED.);
#4417=B_SPLINE_CURVE_WITH_KNOTS('',3,(#175069,#175070,#175071,#175072,#175073,
#175074,#175075,#175076,#175077,#175078,#175079,#175080,#175081,#175082,
#175083,#175084,#175085,#175086,#175087,#175088,#175089,#175090,#175091,
#175092,#175093,#175094,#175095,#175096,#175097,#175098,#175099,#175100,
#175101,#175102,#175103,#175104,#175105),.UNSPECIFIED.,.F.,.F.,(4,3,3,3,
3,3,3,3,3,3,3,3,4),(0.,1.12535551670953E-5,7.76936938401081E-5,0.000102513517961066,
0.00012187918982422,0.000189659041345261,0.000223548967105781,0.000257294099096089,
0.000257438892866301,0.000325720851764136,0.000396486773972714,0.000466242707687174,
0.000514877785732603),.UNSPECIFIED.);
#4418=B_SPLINE_CURVE_WITH_KNOTS('',3,(#175113,#175114,#175115,#175116,#175117,
#175118,#175119,#175120,#175121,#175122,#175123,#175124,#175125,#175126,
#175127,#175128,#175129,#175130,#175131,#175132,#175133,#175134,#175135,
#175136,#175137,#175138,#175139,#175140,#175141,#175142,#175143,#175144,
#175145,#175146,#175147,#175148,#175149,#175150,#175151,#175152),
 .UNSPECIFIED.,.F.,.F.,(4,3,3,3,3,3,3,3,3,3,3,3,3,4),(0.,6.80370855328581E-5,
0.000137303169290931,0.000203636706652317,0.000256396220959702,0.000256540237295726,
0.000285209320207734,0.000342105100635652,0.00038477693595659,0.000400778874201942,
0.000456785658060673,0.000484789049990039,0.000498790745954722,0.000512792441919405),
 .UNSPECIFIED.);
#4419=B_SPLINE_CURVE_WITH_KNOTS('',3,(#175156,#175157,#175158,#175159,#175160,
#175161,#175162,#175163,#175164,#175165,#175166,#175167,#175168,#175169,
#175170,#175171,#175172,#175173,#175174,#175175,#175176,#175177,#175178,
#175179,#175180,#175181,#175182,#175183,#175184,#175185,#175186,#175187,
#175188,#175189,#175190,#175191,#175192),.UNSPECIFIED.,.F.,.F.,(4,3,3,3,
3,3,3,3,3,3,3,3,4),(0.,1.12535551670997E-5,7.76936938475713E-5,0.00010251351796112,
0.000121879189824268,0.000189659041345287,0.000223548967105797,0.000257294099096103,
0.000257438892866306,0.000325720851765822,0.000396486773977161,0.000466242707695556,
0.000514877785732613),.UNSPECIFIED.);
#4420=B_SPLINE_CURVE_WITH_KNOTS('',3,(#175200,#175201,#175202,#175203,#175204,
#175205,#175206,#175207,#175208,#175209,#175210,#175211,#175212,#175213,
#175214,#175215,#175216,#175217,#175218,#175219,#175220,#175221,#175222,
#175223,#175224,#175225,#175226,#175227,#175228,#175229,#175230,#175231,
#175232,#175233,#175234,#175235,#175236,#175237,#175238,#175239),
 .UNSPECIFIED.,.F.,.F.,(4,3,3,3,3,3,3,3,3,3,3,3,3,4),(0.,6.80370855398214E-5,
0.000137303169304995,0.00020363670667273,0.000256396220959706,0.000256540237295733,
0.000285209320207728,0.000342105100635649,0.00038477693595659,0.000400778874201943,
0.000456785658060678,0.000484789049990045,0.000498790745954729,0.000512792441919412),
 .UNSPECIFIED.);
#4421=B_SPLINE_CURVE_WITH_KNOTS('',3,(#175243,#175244,#175245,#175246,#175247,
#175248,#175249,#175250,#175251,#175252,#175253,#175254,#175255,#175256,
#175257,#175258,#175259,#175260,#175261,#175262,#175263,#175264,#175265,
#175266,#175267,#175268,#175269,#175270,#175271,#175272,#175273,#175274,
#175275,#175276,#175277,#175278,#175279),.UNSPECIFIED.,.F.,.F.,(4,3,3,3,
3,3,3,3,3,3,3,3,4),(0.,1.12535551670982E-5,7.76936938418339E-5,0.000102513517961084,
0.000121879189824238,0.000189659041345274,0.000223548967105792,0.000257294099096109,
0.000257438892866311,0.000325720851765796,0.000396486773976165,0.000466242707692333,
0.000514877785732621),.UNSPECIFIED.);
#4422=B_SPLINE_CURVE_WITH_KNOTS('',3,(#175287,#175288,#175289,#175290,#175291,
#175292,#175293,#175294,#175295,#175296,#175297,#175298,#175299,#175300,
#175301,#175302,#175303,#175304,#175305,#175306,#175307,#175308,#175309,
#175310,#175311,#175312,#175313,#175314,#175315,#175316,#175317,#175318,
#175319,#175320,#175321,#175322,#175323,#175324,#175325,#175326),
 .UNSPECIFIED.,.F.,.F.,(4,3,3,3,3,3,3,3,3,3,3,3,3,4),(0.,6.80370855336509E-5,
0.000137303169291916,0.000203636706652182,0.000256396220959706,0.000256540237295742,
0.000285209320207705,0.000342105100635632,0.000384776935956577,0.000400778874201931,
0.000456785658060672,0.000484789049990042,0.000498790745954727,0.000512792441919412),
 .UNSPECIFIED.);
#4423=B_SPLINE_CURVE_WITH_KNOTS('',3,(#175330,#175331,#175332,#175333,#175334,
#175335,#175336,#175337,#175338,#175339,#175340,#175341,#175342,#175343,
#175344,#175345,#175346,#175347,#175348,#175349,#175350,#175351,#175352,
#175353,#175354,#175355,#175356,#175357,#175358,#175359,#175360,#175361,
#175362,#175363,#175364,#175365,#175366),.UNSPECIFIED.,.F.,.F.,(4,3,3,3,
3,3,3,3,3,3,3,3,4),(0.,1.12535551671027E-5,7.76936938492863E-5,0.000102513517961115,
0.000121879189824264,0.000189659041345283,0.000223548967105793,0.000257294099096098,
0.000257438892866303,0.000325720851756605,0.00039648677395862,0.000466242707669241,
0.000514877785732606),.UNSPECIFIED.);
#4424=B_SPLINE_CURVE_WITH_KNOTS('',3,(#175374,#175375,#175376,#175377,#175378,
#175379,#175380,#175381,#175382,#175383,#175384,#175385,#175386,#175387,
#175388,#175389,#175390,#175391,#175392,#175393,#175394,#175395,#175396,
#175397,#175398,#175399,#175400,#175401,#175402,#175403,#175404,#175405,
#175406,#175407,#175408,#175409,#175410,#175411,#175412,#175413),
 .UNSPECIFIED.,.F.,.F.,(4,3,3,3,3,3,3,3,3,3,3,3,3,4),(0.,6.80370855510928E-5,
0.000137303169327734,0.000203636706706446,0.000256396220959707,0.000256540237295735,
0.000285209320207741,0.000342105100635659,0.000384776935956598,0.00040077887420195,
0.000456785658060681,0.000484789049990047,0.00049879074595473,0.000512792441919413),
 .UNSPECIFIED.);
#4425=B_SPLINE_CURVE_WITH_KNOTS('',3,(#175417,#175418,#175419,#175420,#175421,
#175422,#175423,#175424,#175425,#175426,#175427,#175428,#175429,#175430,
#175431,#175432,#175433,#175434,#175435,#175436,#175437,#175438,#175439,
#175440,#175441,#175442,#175443,#175444,#175445,#175446,#175447,#175448,
#175449,#175450,#175451,#175452,#175453),.UNSPECIFIED.,.F.,.F.,(4,3,3,3,
3,3,3,3,3,3,3,3,4),(0.,1.12535551671005E-5,7.7693693864023E-5,0.000102513517961177,
0.000121879189824318,0.000189659041345312,0.000223548967105808,0.000257294099096088,
0.000257438892866305,0.00032572085175239,0.000396486773948841,0.00046624270765219,
0.00051487778573261),.UNSPECIFIED.);
#4426=B_SPLINE_CURVE_WITH_KNOTS('',3,(#175461,#175462,#175463,#175464,#175465,
#175466,#175467,#175468,#175469,#175470,#175471,#175472,#175473,#175474,
#175475,#175476,#175477,#175478,#175479,#175480,#175481,#175482,#175483,
#175484,#175485,#175486,#175487,#175488,#175489,#175490,#175491,#175492,
#175493,#175494,#175495,#175496,#175497,#175498,#175499,#175500),
 .UNSPECIFIED.,.F.,.F.,(4,3,3,3,3,3,3,3,3,3,3,3,3,4),(0.,6.80370855290005E-5,
0.000137303169282125,0.000203636706636526,0.000256396220959704,0.000256540237295738,
0.000285209320207738,0.000342105100635655,0.000384776935956594,0.000400778874201945,
0.000456785658060677,0.000484789049990042,0.000498790745954725,0.000512792441919408),
 .UNSPECIFIED.);
#4427=B_SPLINE_CURVE_WITH_KNOTS('',3,(#175504,#175505,#175506,#175507,#175508,
#175509,#175510,#175511,#175512,#175513,#175514,#175515,#175516,#175517,
#175518,#175519,#175520,#175521,#175522,#175523,#175524,#175525,#175526,
#175527,#175528,#175529,#175530,#175531,#175532,#175533,#175534,#175535,
#175536,#175537,#175538,#175539,#175540),.UNSPECIFIED.,.F.,.F.,(4,3,3,3,
3,3,3,3,3,3,3,3,4),(0.,1.12535551670973E-5,7.76936938483821E-5,0.000102513517961069,
0.000121879189824223,0.000189659041345262,0.000223548967105782,0.000257294099096089,
0.000257438892866301,0.000325720851754469,0.000396486773953083,0.000466242707658755,
0.000514877785732602),.UNSPECIFIED.);
#4428=B_SPLINE_CURVE_WITH_KNOTS('',3,(#175548,#175549,#175550,#175551,#175552,
#175553,#175554,#175555,#175556,#175557,#175558,#175559,#175560,#175561,
#175562,#175563,#175564,#175565,#175566,#175567,#175568,#175569,#175570,
#175571,#175572,#175573,#175574,#175575,#175576,#175577,#175578,#175579,
#175580,#175581,#175582,#175583,#175584,#175585,#175586,#175587),
 .UNSPECIFIED.,.F.,.F.,(4,3,3,3,3,3,3,3,3,3,3,3,3,4),(0.,6.80370855443474E-5,
0.000137303169313637,0.00020363670668462,0.000256396220959708,0.000256540237295739,
0.000285209320207743,0.000342105100635661,0.0003847769359566,0.000400778874201952,
0.000456785658060683,0.000484789049990049,0.000498790745954732,0.000512792441919415),
 .UNSPECIFIED.);
#4429=B_SPLINE_CURVE_WITH_KNOTS('',3,(#175591,#175592,#175593,#175594,#175595,
#175596,#175597,#175598,#175599,#175600,#175601,#175602,#175603,#175604,
#175605,#175606,#175607,#175608,#175609,#175610,#175611,#175612,#175613,
#175614,#175615,#175616,#175617,#175618,#175619,#175620,#175621,#175622,
#175623,#175624,#175625,#175626,#175627),.UNSPECIFIED.,.F.,.F.,(4,3,3,3,
3,3,3,3,3,3,3,3,4),(0.,1.12535551670978E-5,7.76936938552473E-5,0.000102513517961072,
0.000121879189824226,0.000189659041345266,0.000223548967105787,0.000257294099096106,
0.000257438892866307,0.000325720851749875,0.000396486773943902,0.000466242707645584,
0.000514877785732614),.UNSPECIFIED.);
#4430=B_SPLINE_CURVE_WITH_KNOTS('',3,(#175635,#175636,#175637,#175638,#175639,
#175640,#175641,#175642,#175643,#175644,#175645,#175646,#175647,#175648,
#175649,#175650,#175651,#175652,#175653,#175654,#175655,#175656,#175657,
#175658,#175659,#175660,#175661,#175662,#175663,#175664,#175665,#175666,
#175667,#175668,#175669,#175670,#175671,#175672,#175673,#175674),
 .UNSPECIFIED.,.F.,.F.,(4,3,3,3,3,3,3,3,3,3,3,3,3,4),(0.,6.80370855381467E-5,
0.000137303169301509,0.000203636706667771,0.000256396220959704,0.000256540237295722,
0.000285209320207738,0.000342105100635655,0.000384776935956594,0.000400778874201945,
0.000456785658060677,0.000484789049990042,0.000498790745954725,0.000512792441919408),
 .UNSPECIFIED.);
#4431=B_SPLINE_CURVE_WITH_KNOTS('',3,(#175678,#175679,#175680,#175681,#175682,
#175683,#175684,#175685,#175686,#175687,#175688,#175689,#175690,#175691,
#175692,#175693,#175694,#175695,#175696,#175697,#175698,#175699,#175700,
#175701,#175702,#175703,#175704,#175705,#175706,#175707,#175708,#175709,
#175710,#175711,#175712,#175713,#175714),.UNSPECIFIED.,.F.,.F.,(4,3,3,3,
3,3,3,3,3,3,3,3,4),(0.,1.12535551670998E-5,7.76936938400932E-5,0.000102513517961126,
0.000121879189824273,0.000189659041345289,0.000223548967105797,0.000257294099096098,
0.000257438892866305,0.000325720851765772,0.000396486773975871,0.000466242707691754,
0.00051487778573261),.UNSPECIFIED.);
#4432=B_SPLINE_CURVE_WITH_KNOTS('',3,(#175722,#175723,#175724,#175725,#175726,
#175727,#175728,#175729,#175730,#175731,#175732,#175733,#175734,#175735,
#175736,#175737,#175738,#175739,#175740,#175741,#175742,#175743,#175744,
#175745,#175746,#175747,#175748,#175749,#175750,#175751,#175752,#175753,
#175754,#175755,#175756,#175757,#175758,#175759,#175760,#175761),
 .UNSPECIFIED.,.F.,.F.,(4,3,3,3,3,3,3,3,3,3,3,3,3,4),(0.,6.80370855358042E-5,
0.000137303169296868,0.000203636706660701,0.000256396220959706,0.000256540237295732,
0.00028520932020774,0.000342105100635658,0.000384776935956596,0.000400778874201948,
0.00045678565806068,0.000484789049990046,0.000498790745954728,0.000512792441919411),
 .UNSPECIFIED.);
#4433=B_SPLINE_CURVE_WITH_KNOTS('',3,(#175765,#175766,#175767,#175768,#175769,
#175770,#175771,#175772,#175773,#175774,#175775,#175776,#175777,#175778,
#175779,#175780,#175781,#175782,#175783,#175784,#175785,#175786,#175787,
#175788,#175789,#175790,#175791,#175792,#175793,#175794,#175795,#175796,
#175797,#175798,#175799,#175800,#175801),.UNSPECIFIED.,.F.,.F.,(4,3,3,3,
3,3,3,3,3,3,3,3,4),(0.,1.12535551671032E-5,7.76936938466288E-5,0.000102513517961138,
0.000121879189824284,0.000189659041345294,0.000223548967105799,0.000257294099096093,
0.000257438892866304,0.000325720851754854,0.000396486773954175,0.000466242707660958,
0.000514877785732608),.UNSPECIFIED.);
#4434=B_SPLINE_CURVE_WITH_KNOTS('',3,(#175809,#175810,#175811,#175812,#175813,
#175814,#175815,#175816,#175817,#175818,#175819,#175820,#175821,#175822,
#175823,#175824,#175825,#175826,#175827,#175828,#175829,#175830,#175831,
#175832,#175833,#175834,#175835,#175836,#175837,#175838,#175839,#175840,
#175841,#175842,#175843,#175844,#175845,#175846,#175847,#175848),
 .UNSPECIFIED.,.F.,.F.,(4,3,3,3,3,3,3,3,3,3,3,3,3,4),(0.,6.8037085539341E-5,
0.000137303169304,0.000203636706671485,0.000256396220959705,0.000256540237295733,
0.000285209320207739,0.000342105100635656,0.000384776935956594,0.000400778874201946,
0.000456785658060678,0.000484789049990043,0.000498790745954726,0.000512792441919409),
 .UNSPECIFIED.);
#4435=B_SPLINE_CURVE_WITH_KNOTS('',3,(#175855,#175856,#175857,#175858,#175859,
#175860,#175861,#175862,#175863,#175864,#175865,#175866,#175867,#175868,
#175869,#175870,#175871,#175872,#175873,#175874,#175875,#175876,#175877,
#175878,#175879,#175880,#175881,#175882,#175883,#175884,#175885,#175886,
#175887,#175888,#175889,#175890,#175891),.UNSPECIFIED.,.F.,.F.,(4,3,3,3,
3,3,3,3,3,3,3,3,4),(0.,1.12535551671012E-5,7.76936938518268E-5,0.000102513517961145,
0.00012187918982429,0.000189659041345297,0.000223548967105801,0.000257294099096108,
0.000257438892866305,0.000325720851757891,0.000396486773960361,0.000466242707669812,
0.00051487778573261),.UNSPECIFIED.);
#4436=B_SPLINE_CURVE_WITH_KNOTS('',3,(#175899,#175900,#175901,#175902,#175903,
#175904,#175905,#175906,#175907,#175908,#175909,#175910,#175911,#175912,
#175913,#175914,#175915,#175916,#175917,#175918,#175919,#175920,#175921,
#175922,#175923,#175924,#175925,#175926,#175927,#175928,#175929,#175930,
#175931,#175932,#175933,#175934,#175935,#175936,#175937,#175938),
 .UNSPECIFIED.,.F.,.F.,(4,3,3,3,3,3,3,3,3,3,3,3,3,4),(0.,6.8037085541032E-5,
0.000137303169307532,0.000203636706676779,0.000256396220959702,0.00025654023729573,
0.000285209320207736,0.000342105100635653,0.000384776935956591,0.000400778874201943,
0.000456785658060674,0.000484789049990039,0.000498790745954722,0.000512792441919405),
 .UNSPECIFIED.);
#4437=B_SPLINE_CURVE_WITH_KNOTS('',3,(#175942,#175943,#175944,#175945,#175946,
#175947,#175948,#175949,#175950,#175951,#175952,#175953,#175954,#175955,
#175956,#175957,#175958,#175959,#175960,#175961,#175962,#175963,#175964,
#175965,#175966,#175967,#175968,#175969,#175970,#175971,#175972,#175973,
#175974,#175975,#175976,#175977,#175978),.UNSPECIFIED.,.F.,.F.,(4,3,3,3,
3,3,3,3,3,3,3,3,4),(0.,1.1253555167099E-5,7.76936938452608E-5,0.000102513517961139,
0.000121879189824284,0.000189659041345294,0.000223548967105799,0.00025729409909611,
0.000257438892866304,0.000325720851760016,0.000396486773964437,0.000466242707675329,
0.000514877785732608),.UNSPECIFIED.);
#4438=B_SPLINE_CURVE_WITH_KNOTS('',3,(#175986,#175987,#175988,#175989,#175990,
#175991,#175992,#175993,#175994,#175995,#175996,#175997,#175998,#175999,
#176000,#176001,#176002,#176003,#176004,#176005,#176006,#176007,#176008,
#176009,#176010,#176011,#176012,#176013,#176014,#176015,#176016,#176017,
#176018,#176019,#176020,#176021,#176022,#176023,#176024,#176025),
 .UNSPECIFIED.,.F.,.F.,(4,3,3,3,3,3,3,3,3,3,3,3,3,4),(0.,6.80370855344135E-5,
0.000137303169294105,0.000203636706657015,0.000256396220959704,0.000256540237295728,
0.000285209320207741,0.000342105100635657,0.000384776935956595,0.000400778874201946,
0.000456785658060677,0.000484789049990042,0.000498790745954725,0.000512792441919407),
 .UNSPECIFIED.);
#4439=B_SPLINE_CURVE_WITH_KNOTS('',3,(#176029,#176030,#176031,#176032,#176033,
#176034,#176035,#176036,#176037,#176038,#176039,#176040,#176041,#176042,
#176043,#176044,#176045,#176046,#176047,#176048,#176049,#176050,#176051,
#176052,#176053,#176054,#176055,#176056,#176057,#176058,#176059,#176060,
#176061,#176062,#176063,#176064,#176065),.UNSPECIFIED.,.F.,.F.,(4,3,3,3,
3,3,3,3,3,3,3,3,4),(0.,1.12535551670998E-5,7.76936938473757E-5,0.000102513517961127,
0.000121879189824274,0.000189659041345289,0.000223548967105796,0.000257294099096108,
0.000257438892866304,0.000325720851760781,0.000396486773966304,0.000466242707678675,
0.000514877785732608),.UNSPECIFIED.);
#4440=B_SPLINE_CURVE_WITH_KNOTS('',3,(#176073,#176074,#176075,#176076,#176077,
#176078,#176079,#176080,#176081,#176082,#176083,#176084,#176085,#176086,
#176087,#176088,#176089,#176090,#176091,#176092,#176093,#176094,#176095,
#176096,#176097,#176098,#176099,#176100,#176101,#176102,#176103,#176104,
#176105,#176106,#176107,#176108,#176109,#176110,#176111,#176112),
 .UNSPECIFIED.,.F.,.F.,(4,3,3,3,3,3,3,3,3,3,3,3,3,4),(0.,6.80370855324475E-5,
0.000137303169290076,0.000203636706650847,0.000256396220959707,0.000256540237295739,
0.000285209320207734,0.000342105100635654,0.000384776935956594,0.000400778874201946,
0.00045678565806068,0.000484789049990047,0.00049879074595473,0.000512792441919413),
 .UNSPECIFIED.);
#4441=B_SPLINE_CURVE_WITH_KNOTS('',3,(#176116,#176117,#176118,#176119,#176120,
#176121,#176122,#176123,#176124,#176125,#176126,#176127,#176128,#176129,
#176130,#176131,#176132,#176133,#176134,#176135,#176136,#176137,#176138,
#176139,#176140,#176141,#176142,#176143,#176144,#176145,#176146,#176147,
#176148,#176149,#176150,#176151,#176152),.UNSPECIFIED.,.F.,.F.,(4,3,3,3,
3,3,3,3,3,3,3,3,4),(0.,1.12535551671022E-5,7.7693693845666E-5,0.00010251351796117,
0.000121879189824311,0.000189659041345307,0.000223548967105805,0.000257294099096107,
0.000257438892866303,0.00032572085175553,0.000396486773955308,0.00046624270766216,
0.000514877785732605),.UNSPECIFIED.);
#4442=B_SPLINE_CURVE_WITH_KNOTS('',3,(#176160,#176161,#176162,#176163,#176164,
#176165,#176166,#176167,#176168,#176169,#176170,#176171,#176172,#176173,
#176174,#176175,#176176,#176177,#176178,#176179,#176180,#176181,#176182,
#176183,#176184,#176185,#176186,#176187,#176188,#176189,#176190,#176191,
#176192,#176193,#176194,#176195,#176196,#176197,#176198,#176199),
 .UNSPECIFIED.,.F.,.F.,(4,3,3,3,3,3,3,3,3,3,3,3,3,4),(0.,6.8037085543224E-5,
0.000137303169311952,0.000203636706683699,0.000256396220959705,0.000256540237295732,
0.000285209320207731,0.00034210510063565,0.00038477693595659,0.000400778874201943,
0.000456785658060676,0.000484789049990043,0.000498790745954727,0.00051279244191941),
 .UNSPECIFIED.);
#4443=B_SPLINE_CURVE_WITH_KNOTS('',3,(#176203,#176204,#176205,#176206,#176207,
#176208,#176209,#176210,#176211,#176212,#176213,#176214,#176215,#176216,
#176217,#176218,#176219,#176220,#176221,#176222,#176223,#176224,#176225,
#176226,#176227,#176228,#176229,#176230,#176231,#176232,#176233,#176234,
#176235,#176236,#176237,#176238,#176239),.UNSPECIFIED.,.F.,.F.,(4,3,3,3,
3,3,3,3,3,3,3,3,4),(0.,1.12535551671005E-5,7.7693693841547E-5,0.000102513517961162,
0.000121879189824305,0.000189659041345307,0.000223548967105808,0.000257294099096097,
0.000257438892866309,0.000325720851762212,0.000396486773968726,0.000466242707681267,
0.000514877785732617),.UNSPECIFIED.);
#4444=B_SPLINE_CURVE_WITH_KNOTS('',3,(#176247,#176248,#176249,#176250,#176251,
#176252,#176253,#176254,#176255,#176256,#176257,#176258,#176259,#176260,
#176261,#176262,#176263,#176264,#176265,#176266,#176267,#176268,#176269,
#176270,#176271,#176272,#176273,#176274,#176275,#176276,#176277,#176278,
#176279,#176280,#176281,#176282,#176283,#176284,#176285,#176286),
 .UNSPECIFIED.,.F.,.F.,(4,3,3,3,3,3,3,3,3,3,3,3,3,4),(0.,6.80370855366589E-5,
0.000137303169298556,0.00020363670666332,0.000256396220959708,0.000256540237295731,
0.000285209320207723,0.000342105100635647,0.000384776935956589,0.000400778874201942,
0.000456785658060679,0.000484789049990048,0.000498790745954732,0.000512792441919417),
 .UNSPECIFIED.);
#4445=B_SPLINE_CURVE_WITH_KNOTS('',3,(#176290,#176291,#176292,#176293,#176294,
#176295,#176296,#176297,#176298,#176299,#176300,#176301,#176302,#176303,
#176304,#176305,#176306,#176307,#176308,#176309,#176310,#176311,#176312,
#176313,#176314,#176315,#176316,#176317,#176318,#176319,#176320,#176321,
#176322,#176323,#176324,#176325,#176326),.UNSPECIFIED.,.F.,.F.,(4,3,3,3,
3,3,3,3,3,3,3,3,4),(0.,1.12535551670983E-5,7.76936938510176E-5,0.000102513517961093,
0.000121879189824245,0.000189659041345275,0.00022354896710579,0.000257294099096106,
0.000257438892866305,0.00032572085175851,0.000396486773961158,0.000466242707670101,
0.0005148777857326),.UNSPECIFIED.);
#4446=B_SPLINE_CURVE_WITH_KNOTS('',3,(#176334,#176335,#176336,#176337,#176338,
#176339,#176340,#176341,#176342,#176343,#176344,#176345,#176346,#176347,
#176348,#176349,#176350,#176351,#176352,#176353,#176354,#176355,#176356,
#176357,#176358,#176359,#176360,#176361,#176362,#176363,#176364,#176365,
#176366,#176367,#176368,#176369,#176370,#176371,#176372,#176373),
 .UNSPECIFIED.,.F.,.F.,(4,3,3,3,3,3,3,3,3,3,3,3,3,4),(0.,6.80370855381278E-5,
0.000137303169302431,0.000203636706670777,0.000256396220959703,0.000256540237295731,
0.000285209320207733,0.000342105100635651,0.00038477693595659,0.000400778874201942,
0.000456785658060674,0.00048478904999004,0.000498790745954723,0.000512792441919405),
 .UNSPECIFIED.);
#4447=B_SPLINE_CURVE_WITH_KNOTS('',3,(#176377,#176378,#176379,#176380,#176381,
#176382,#176383,#176384,#176385,#176386,#176387,#176388,#176389,#176390,
#176391,#176392,#176393,#176394,#176395,#176396,#176397,#176398,#176399,
#176400,#176401,#176402,#176403,#176404,#176405,#176406,#176407,#176408,
#176409,#176410,#176411,#176412,#176413),.UNSPECIFIED.,.F.,.F.,(4,3,3,3,
3,3,3,3,3,3,3,3,4),(0.,1.12535551671016E-5,7.76936938479796E-5,0.000102513517961101,
0.000121879189824252,0.000189659041345279,0.000223548967105792,0.000257294099096099,
0.000257438892866305,0.000325720851745948,0.000396486773936273,0.000466242707635578,
0.000514877785732611),.UNSPECIFIED.);
#4448=B_SPLINE_CURVE_WITH_KNOTS('',3,(#176421,#176422,#176423,#176424,#176425,
#176426,#176427,#176428,#176429,#176430,#176431,#176432,#176433,#176434,
#176435,#176436,#176437,#176438,#176439,#176440,#176441,#176442,#176443,
#176444,#176445,#176446,#176447,#176448,#176449,#176450,#176451,#176452,
#176453,#176454,#176455,#176456,#176457,#176458,#176459,#176460),
 .UNSPECIFIED.,.F.,.F.,(4,3,3,3,3,3,3,3,3,3,3,3,3,4),(0.,6.80370855407977E-5,
0.0001373031693065,0.00020363670667411,0.000256396220959709,0.00025654023729572,
0.000285209320207748,0.000342105100635665,0.000384776935956604,0.000400778874201955,
0.000456785658060687,0.000484789049990053,0.000498790745954735,0.000512792441919418),
 .UNSPECIFIED.);
#4449=B_SPLINE_CURVE_WITH_KNOTS('',3,(#176464,#176465,#176466,#176467,#176468,
#176469,#176470,#176471,#176472,#176473,#176474,#176475,#176476,#176477,
#176478,#176479,#176480,#176481,#176482,#176483,#176484,#176485,#176486,
#176487,#176488,#176489,#176490,#176491,#176492,#176493,#176494,#176495,
#176496,#176497,#176498,#176499,#176500),.UNSPECIFIED.,.F.,.F.,(4,3,3,3,
3,3,3,3,3,3,3,3,4),(0.,1.12535551671054E-5,7.76936938616112E-5,0.000102513517961212,
0.000121879189824349,0.000189659041345329,0.00022354896710582,0.00025729409909611,
0.00025743889286631,0.000325720851754512,0.000396486773953998,0.000466242707661241,
0.00051487778573262),.UNSPECIFIED.);
#4450=B_SPLINE_CURVE_WITH_KNOTS('',3,(#176508,#176509,#176510,#176511,#176512,
#176513,#176514,#176515,#176516,#176517,#176518,#176519,#176520,#176521,
#176522,#176523,#176524,#176525,#176526,#176527,#176528,#176529,#176530,
#176531,#176532,#176533,#176534,#176535,#176536,#176537,#176538,#176539,
#176540,#176541,#176542,#176543,#176544,#176545,#176546,#176547),
 .UNSPECIFIED.,.F.,.F.,(4,3,3,3,3,3,3,3,3,3,3,3,3,4),(0.,6.80370855414931E-5,
0.000137303169307904,0.000203636706675899,0.000256396220959702,0.000256540237295727,
0.00028520932020771,0.000342105100635634,0.000384776935956576,0.00040077887420193,
0.000456785658060667,0.000484789049990036,0.00049879074595472,0.000512792441919405),
 .UNSPECIFIED.);
#4451=B_SPLINE_CURVE_WITH_KNOTS('',3,(#176551,#176552,#176553,#176554,#176555,
#176556,#176557,#176558,#176559,#176560,#176561,#176562,#176563,#176564,
#176565,#176566,#176567,#176568,#176569,#176570,#176571,#176572,#176573,
#176574,#176575,#176576,#176577,#176578,#176579,#176580,#176581,#176582,
#176583,#176584,#176585,#176586,#176587),.UNSPECIFIED.,.F.,.F.,(4,3,3,3,
3,3,3,3,3,3,3,3,4),(0.,1.12535551671044E-5,7.76936938352556E-5,0.000102513517961147,
0.000121879189824292,0.000189659041345301,0.000223548967105805,0.000257294099096117,
0.00025743889286631,0.000325720851753075,0.000396486773950483,0.000466242707655942,
0.000514877785732619),.UNSPECIFIED.);
#4452=B_SPLINE_CURVE_WITH_KNOTS('',3,(#176595,#176596,#176597,#176598,#176599,
#176600,#176601,#176602,#176603,#176604,#176605,#176606,#176607,#176608,
#176609,#176610,#176611,#176612,#176613,#176614,#176615,#176616,#176617,
#176618,#176619,#176620,#176621,#176622,#176623,#176624,#176625,#176626,
#176627,#176628,#176629,#176630,#176631,#176632,#176633,#176634),
 .UNSPECIFIED.,.F.,.F.,(4,3,3,3,3,3,3,3,3,3,3,3,3,4),(0.,6.80370855377875E-5,
0.000137303169301054,0.000203636706667488,0.000256396220959705,0.00025654023729572,
0.000285209320207726,0.000342105100635647,0.000384776935956588,0.00040077887420194,
0.000456785658060675,0.000484789049990043,0.000498790745954726,0.00051279244191941),
 .UNSPECIFIED.);
#4453=B_SPLINE_CURVE_WITH_KNOTS('',3,(#176638,#176639,#176640,#176641,#176642,
#176643,#176644,#176645,#176646,#176647,#176648,#176649,#176650,#176651,
#176652,#176653,#176654,#176655,#176656,#176657,#176658,#176659,#176660,
#176661,#176662,#176663,#176664,#176665,#176666,#176667,#176668,#176669,
#176670,#176671,#176672,#176673,#176674),.UNSPECIFIED.,.F.,.F.,(4,3,3,3,
3,3,3,3,3,3,3,3,4),(0.,1.12535551671036E-5,7.76936938472083E-5,0.000102513517961145,
0.00012187918982429,0.000189659041345296,0.000223548967105799,0.000257294099096105,
0.000257438892866302,0.000325720851742521,0.000396486773928871,0.000466242707623768,
0.000514877785732603),.UNSPECIFIED.);
#4454=B_SPLINE_CURVE_WITH_KNOTS('',3,(#176682,#176683,#176684,#176685,#176686,
#176687,#176688,#176689,#176690,#176691,#176692,#176693,#176694,#176695,
#176696,#176697,#176698,#176699,#176700,#176701,#176702,#176703,#176704,
#176705,#176706,#176707,#176708,#176709,#176710,#176711,#176712,#176713,
#176714,#176715,#176716,#176717,#176718,#176719,#176720,#176721),
 .UNSPECIFIED.,.F.,.F.,(4,3,3,3,3,3,3,3,3,3,3,3,3,4),(0.,6.80370855369261E-5,
0.000137303169298902,0.000203636706663393,0.000256396220959703,0.000256540237295733,
0.000285209320207716,0.000342105100635638,0.00038477693595658,0.000400778874201934,
0.00045678565806067,0.000484789049990038,0.000498790745954722,0.000512792441919406),
 .UNSPECIFIED.);
#4455=B_SPLINE_CURVE_WITH_KNOTS('',3,(#176725,#176726,#176727,#176728,#176729,
#176730,#176731,#176732,#176733,#176734,#176735,#176736,#176737,#176738,
#176739,#176740,#176741,#176742,#176743,#176744,#176745,#176746,#176747,
#176748,#176749,#176750,#176751,#176752,#176753,#176754,#176755,#176756,
#176757,#176758,#176759,#176760,#176761),.UNSPECIFIED.,.F.,.F.,(4,3,3,3,
3,3,3,3,3,3,3,3,4),(0.,1.12535551670904E-5,7.76936938439903E-5,0.00010251351796104,
0.000121879189824199,0.000189659041345254,0.000223548967105781,0.000257294099096101,
0.000257438892866308,0.000325720851761651,0.000396486773967453,0.000466242707679148,
0.000514877785732617),.UNSPECIFIED.);
#4456=B_SPLINE_CURVE_WITH_KNOTS('',3,(#176769,#176770,#176771,#176772,#176773,
#176774,#176775,#176776,#176777,#176778,#176779,#176780,#176781,#176782,
#176783,#176784,#176785,#176786,#176787,#176788,#176789,#176790,#176791,
#176792,#176793,#176794,#176795,#176796,#176797,#176798,#176799,#176800,
#176801,#176802,#176803,#176804,#176805,#176806,#176807,#176808),
 .UNSPECIFIED.,.F.,.F.,(4,3,3,3,3,3,3,3,3,3,3,3,3,4),(0.,6.80370855361831E-5,
0.000137303169297157,0.000203636706660255,0.000256396220959701,0.000256540237295729,
0.000285209320207742,0.000342105100635657,0.000384776935956594,0.000400778874201945,
0.000456785658060674,0.000484789049990038,0.00049879074595472,0.000512792441919403),
 .UNSPECIFIED.);
#4457=B_SPLINE_CURVE_WITH_KNOTS('',3,(#176812,#176813,#176814,#176815,#176816,
#176817,#176818,#176819,#176820,#176821,#176822,#176823,#176824,#176825,
#176826,#176827,#176828,#176829,#176830,#176831,#176832,#176833,#176834,
#176835,#176836,#176837,#176838,#176839,#176840,#176841,#176842,#176843,
#176844,#176845,#176846,#176847,#176848),.UNSPECIFIED.,.F.,.F.,(4,3,3,3,
3,3,3,3,3,3,3,3,4),(0.,1.12535551671015E-5,7.76936938530422E-5,0.00010251351796114,
0.000121879189824285,0.00018965904134529,0.000223548967105792,0.000257294099096101,
0.000257438892866295,0.000325720851754998,0.000396486773954111,0.000466242707659906,
0.00051487778573259),.UNSPECIFIED.);
#4458=B_SPLINE_CURVE_WITH_KNOTS('',3,(#176856,#176857,#176858,#176859,#176860,
#176861,#176862,#176863,#176864,#176865,#176866,#176867,#176868,#176869,
#176870,#176871,#176872,#176873,#176874,#176875,#176876,#176877,#176878,
#176879,#176880,#176881,#176882,#176883,#176884,#176885,#176886,#176887,
#176888,#176889,#176890,#176891,#176892,#176893,#176894,#176895),
 .UNSPECIFIED.,.F.,.F.,(4,3,3,3,3,3,3,3,3,3,3,3,3,4),(0.,6.80370855425714E-5,
0.000137303169310326,0.000203636706679929,0.000256396220959705,0.000256540237295739,
0.000285209320207736,0.000342105100635654,0.000384776935956593,0.000400778874201945,
0.000456785658060677,0.000484789049990043,0.000498790745954727,0.00051279244191941),
 .UNSPECIFIED.);
#4459=B_SPLINE_CURVE_WITH_KNOTS('',3,(#176899,#176900,#176901,#176902,#176903,
#176904,#176905,#176906,#176907,#176908,#176909,#176910,#176911,#176912,
#176913,#176914,#176915,#176916,#176917,#176918,#176919,#176920,#176921,
#176922,#176923,#176924,#176925,#176926,#176927,#176928,#176929,#176930,
#176931,#176932,#176933,#176934,#176935),.UNSPECIFIED.,.F.,.F.,(4,3,3,3,
3,3,3,3,3,3,3,3,4),(0.,1.12535551670989E-5,7.76936938471546E-5,0.00010251351796113,
0.000121879189824276,0.00018965904134529,0.000223548967105796,0.00025729409909611,
0.000257438892866303,0.000325720851757156,0.000396486773958549,0.000466242707666787,
0.000514877785732606),.UNSPECIFIED.);
#4460=B_SPLINE_CURVE_WITH_KNOTS('',3,(#176943,#176944,#176945,#176946,#176947,
#176948,#176949,#176950,#176951,#176952,#176953,#176954,#176955,#176956,
#176957,#176958,#176959,#176960,#176961,#176962,#176963,#176964,#176965,
#176966,#176967,#176968,#176969,#176970,#176971,#176972,#176973,#176974,
#176975,#176976,#176977,#176978,#176979,#176980,#176981,#176982),
 .UNSPECIFIED.,.F.,.F.,(4,3,3,3,3,3,3,3,3,3,3,3,3,4),(0.,6.80370855337926E-5,
0.000137303169293006,0.00020363670665551,0.000256396220959705,0.000256540237295733,
0.000285209320207729,0.000342105100635649,0.000384776935956589,0.000400778874201942,
0.000456785658060675,0.000484789049990042,0.000498790745954726,0.000512792441919409),
 .UNSPECIFIED.);
#4461=B_SPLINE_CURVE_WITH_KNOTS('',3,(#176986,#176987,#176988,#176989,#176990,
#176991,#176992,#176993,#176994,#176995,#176996,#176997,#176998,#176999,
#177000,#177001,#177002,#177003,#177004,#177005,#177006,#177007,#177008,
#177009,#177010,#177011,#177012,#177013,#177014,#177015,#177016,#177017,
#177018,#177019,#177020,#177021,#177022),.UNSPECIFIED.,.F.,.F.,(4,3,3,3,
3,3,3,3,3,3,3,3,4),(0.,1.12535551671055E-5,7.76936938444389E-5,0.000102513517961177,
0.000121879189824318,0.000189659041345312,0.000223548967105809,0.000257294099096115,
0.000257438892866307,0.000325720851758166,0.000396486773960672,0.00046624270767006,
0.000514877785732613),.UNSPECIFIED.);
#4462=B_SPLINE_CURVE_WITH_KNOTS('',3,(#177030,#177031,#177032,#177033,#177034,
#177035,#177036,#177037,#177038,#177039,#177040,#177041,#177042,#177043,
#177044,#177045,#177046,#177047,#177048,#177049,#177050,#177051,#177052,
#177053,#177054,#177055,#177056,#177057,#177058,#177059,#177060,#177061,
#177062,#177063,#177064,#177065,#177066,#177067,#177068,#177069),
 .UNSPECIFIED.,.F.,.F.,(4,3,3,3,3,3,3,3,3,3,3,3,3,4),(0.,6.80370855295494E-5,
0.000137303169284071,0.000203636706641568,0.000256396220959705,0.000256540237295731,
0.000285209320207737,0.000342105100635655,0.000384776935956594,0.000400778874201946,
0.000456785658060678,0.000484789049990043,0.000498790745954726,0.000512792441919409),
 .UNSPECIFIED.);
#4463=B_SPLINE_CURVE_WITH_KNOTS('',3,(#177073,#177074,#177075,#177076,#177077,
#177078,#177079,#177080,#177081,#177082,#177083,#177084,#177085,#177086,
#177087,#177088,#177089,#177090,#177091,#177092,#177093,#177094,#177095,
#177096,#177097,#177098,#177099,#177100,#177101,#177102,#177103,#177104,
#177105,#177106,#177107,#177108,#177109),.UNSPECIFIED.,.F.,.F.,(4,3,3,3,
3,3,3,3,3,3,3,3,4),(0.,1.12535551670975E-5,7.76936938472089E-5,0.000102513517961106,
0.000121879189824256,0.00018965904134528,0.000223548967105792,0.000257294099096117,
0.000257438892866304,0.000325720851759813,0.000396486773964141,0.000466242707675212,
0.000514877785732608),.UNSPECIFIED.);
#4464=B_SPLINE_CURVE_WITH_KNOTS('',3,(#177116,#177117,#177118,#177119,#177120,
#177121,#177122,#177123,#177124,#177125,#177126,#177127,#177128,#177129,
#177130,#177131,#177132,#177133,#177134,#177135,#177136,#177137,#177138,
#177139,#177140,#177141,#177142,#177143,#177144,#177145,#177146,#177147,
#177148,#177149,#177150,#177151,#177152,#177153,#177154,#177155),
 .UNSPECIFIED.,.F.,.F.,(4,3,3,3,3,3,3,3,3,3,3,3,3,4),(0.,6.80370855426575E-5,
0.000137303169310749,0.000203636706681619,0.000256396220959708,0.00025654023729573,
0.000285209320207732,0.000342105100635653,0.000384776935956594,0.000400778874201947,
0.000456785658060682,0.000484789049990049,0.000498790745954733,0.000512792441919416),
 .UNSPECIFIED.);
#4465=B_SPLINE_CURVE_WITH_KNOTS('',3,(#177157,#177158,#177159,#177160,#177161,
#177162,#177163,#177164,#177165,#177166,#177167,#177168,#177169,#177170,
#177171,#177172,#177173,#177174,#177175,#177176,#177177,#177178,#177179,
#177180,#177181,#177182,#177183,#177184,#177185,#177186,#177187,#177188,
#177189,#177190,#177191,#177192,#177193),.UNSPECIFIED.,.F.,.F.,(4,3,3,3,
3,3,3,3,3,3,3,3,4),(0.,1.12535551670974E-5,7.76936938451676E-5,0.000102513517961093,
0.000121879189824244,0.000189659041345273,0.000223548967105788,0.000257294099096101,
0.000257438892866302,0.000325720851758372,0.000396486773961206,0.000466242707671043,
0.000514877785732605),.UNSPECIFIED.);
#4466=B_SPLINE_CURVE_WITH_KNOTS('',3,(#177201,#177202,#177203,#177204,#177205,
#177206,#177207,#177208,#177209,#177210,#177211,#177212,#177213,#177214,
#177215,#177216,#177217,#177218,#177219,#177220,#177221,#177222,#177223,
#177224,#177225,#177226,#177227,#177228,#177229,#177230,#177231,#177232,
#177233,#177234,#177235,#177236,#177237,#177238,#177239,#177240),
 .UNSPECIFIED.,.F.,.F.,(4,3,3,3,3,3,3,3,3,3,3,3,3,4),(0.,6.80370855381835E-5,
0.000137303169301825,0.000203636706668595,0.000256396220959707,0.00025654023729572,
0.000285209320207731,0.000342105100635652,0.000384776935956593,0.000400778874201946,
0.00045678565806068,0.000484789049990048,0.000498790745954731,0.000512792441919415),
 .UNSPECIFIED.);
#4467=B_SPLINE_CURVE_WITH_KNOTS('',3,(#177244,#177245,#177246,#177247,#177248,
#177249,#177250,#177251,#177252,#177253,#177254,#177255,#177256,#177257,
#177258,#177259,#177260,#177261,#177262,#177263,#177264,#177265,#177266,
#177267,#177268,#177269,#177270,#177271,#177272,#177273,#177274,#177275,
#177276,#177277,#177278,#177279,#177280),.UNSPECIFIED.,.F.,.F.,(4,3,3,3,
3,3,3,3,3,3,3,3,4),(0.,1.12535551670995E-5,7.76936938489843E-5,0.000102513517961118,
0.000121879189824266,0.000189659041345285,0.000223548967105795,0.000257294099096108,
0.000257438892866304,0.00032572085175959,0.00039648677396363,0.000466242707674216,
0.000514877785732608),.UNSPECIFIED.);
#4468=B_SPLINE_CURVE_WITH_KNOTS('',3,(#177288,#177289,#177290,#177291,#177292,
#177293,#177294,#177295,#177296,#177297,#177298,#177299,#177300,#177301,
#177302,#177303,#177304,#177305,#177306,#177307,#177308,#177309,#177310,
#177311,#177312,#177313,#177314,#177315,#177316,#177317,#177318,#177319,
#177320,#177321,#177322,#177323,#177324,#177325,#177326,#177327),
 .UNSPECIFIED.,.F.,.F.,(4,3,3,3,3,3,3,3,3,3,3,3,3,4),(0.,6.80370855408551E-5,
0.000137303169307171,0.000203636706676362,0.000256396220959704,0.00025654023729573,
0.000285209320207735,0.000342105100635653,0.000384776935956592,0.000400778874201944,
0.000456785658060676,0.000484789049990042,0.000498790745954725,0.000512792441919408),
 .UNSPECIFIED.);
#4469=B_SPLINE_CURVE_WITH_KNOTS('',3,(#177331,#177332,#177333,#177334,#177335,
#177336,#177337,#177338,#177339,#177340,#177341,#177342,#177343,#177344,
#177345,#177346,#177347,#177348,#177349,#177350,#177351,#177352,#177353,
#177354,#177355,#177356,#177357,#177358,#177359,#177360,#177361,#177362,
#177363,#177364,#177365,#177366,#177367),.UNSPECIFIED.,.F.,.F.,(4,3,3,3,
3,3,3,3,3,3,3,3,4),(0.,1.12535551671002E-5,7.7693693839773E-5,0.000102513517961098,
0.000121879189824249,0.000189659041345276,0.00022354896710579,0.000257294099096113,
0.000257438892866304,0.00032572085175236,0.000396486773948729,0.000466242707652564,
0.000514877785732609),.UNSPECIFIED.);
#4470=B_SPLINE_CURVE_WITH_KNOTS('',3,(#177375,#177376,#177377,#177378,#177379,
#177380,#177381,#177382,#177383,#177384,#177385,#177386,#177387,#177388,
#177389,#177390,#177391,#177392,#177393,#177394,#177395,#177396,#177397,
#177398,#177399,#177400,#177401,#177402,#177403,#177404,#177405,#177406,
#177407,#177408,#177409,#177410,#177411,#177412,#177413,#177414),
 .UNSPECIFIED.,.F.,.F.,(4,3,3,3,3,3,3,3,3,3,3,3,3,4),(0.,6.80370855356796E-5,
0.000137303169296129,0.000203636706658719,0.000256396220959703,0.000256540237295748,
0.00028520932020774,0.000342105100635656,0.000384776935956594,0.000400778874201945,
0.000456785658060676,0.000484789049990041,0.000498790745954723,0.000512792441919406),
 .UNSPECIFIED.);
#4471=B_SPLINE_CURVE_WITH_KNOTS('',3,(#177418,#177419,#177420,#177421,#177422,
#177423,#177424,#177425,#177426,#177427,#177428,#177429,#177430,#177431,
#177432,#177433,#177434,#177435,#177436,#177437,#177438,#177439,#177440,
#177441,#177442,#177443,#177444,#177445,#177446,#177447,#177448,#177449,
#177450,#177451,#177452,#177453,#177454),.UNSPECIFIED.,.F.,.F.,(4,3,3,3,
3,3,3,3,3,3,3,3,4),(0.,1.12535551670962E-5,7.76936938524064E-5,0.000102513517961067,
0.000121879189824222,0.000189659041345266,0.000223548967105787,0.000257294099096103,
0.000257438892866309,0.000325720851742739,0.000396486773928982,0.000466242707623088,
0.000514877785732618),.UNSPECIFIED.);
#4472=B_SPLINE_CURVE_WITH_KNOTS('',3,(#177462,#177463,#177464,#177465,#177466,
#177467,#177468,#177469,#177470,#177471,#177472,#177473,#177474,#177475,
#177476,#177477,#177478,#177479,#177480,#177481,#177482,#177483,#177484,
#177485,#177486,#177487,#177488,#177489,#177490,#177491,#177492,#177493,
#177494,#177495,#177496,#177497,#177498,#177499,#177500,#177501),
 .UNSPECIFIED.,.F.,.F.,(4,3,3,3,3,3,3,3,3,3,3,3,3,4),(0.,6.8037085537137E-5,
0.000137303169299574,0.000203636706665128,0.000256396220959701,0.000256540237295749,
0.000285209320207748,0.000342105100635662,0.000384776935956597,0.000400778874201948,
0.000456785658060675,0.000484789049990039,0.000498790745954721,0.000512792441919403),
 .UNSPECIFIED.);
#4473=B_SPLINE_CURVE_WITH_KNOTS('',3,(#177505,#177506,#177507,#177508,#177509,
#177510,#177511,#177512,#177513,#177514,#177515,#177516,#177517,#177518,
#177519,#177520,#177521,#177522,#177523,#177524,#177525,#177526,#177527,
#177528,#177529,#177530,#177531,#177532,#177533,#177534,#177535,#177536,
#177537,#177538,#177539,#177540,#177541),.UNSPECIFIED.,.F.,.F.,(4,3,3,3,
3,3,3,3,3,3,3,3,4),(0.,1.12535551670965E-5,7.76936938401387E-5,0.000102513517961103,
0.000121879189824253,0.00018965904134528,0.000223548967105793,0.000257294099096109,
0.000257438892866306,0.000325720851768072,0.000396486773980999,0.00046624270769989,
0.000514877785732612),.UNSPECIFIED.);
#4474=B_SPLINE_CURVE_WITH_KNOTS('',3,(#177549,#177550,#177551,#177552,#177553,
#177554,#177555,#177556,#177557,#177558,#177559,#177560,#177561,#177562,
#177563,#177564,#177565,#177566,#177567,#177568,#177569,#177570,#177571,
#177572,#177573,#177574,#177575,#177576,#177577,#177578,#177579,#177580,
#177581,#177582,#177583,#177584,#177585,#177586,#177587,#177588),
 .UNSPECIFIED.,.F.,.F.,(4,3,3,3,3,3,3,3,3,3,3,3,3,4),(0.,6.80370855398071E-5,
0.000137303169305327,0.000203636706674421,0.000256396220959704,0.000256540237295728,
0.000285209320207732,0.000342105100635651,0.00038477693595659,0.000400778874201942,
0.000456785658060675,0.000484789049990041,0.000498790745954725,0.000512792441919408),
 .UNSPECIFIED.);
#4475=B_SPLINE_CURVE_WITH_KNOTS('',3,(#177592,#177593,#177594,#177595,#177596,
#177597,#177598,#177599,#177600,#177601,#177602,#177603,#177604,#177605,
#177606,#177607,#177608,#177609,#177610,#177611,#177612,#177613,#177614,
#177615,#177616,#177617,#177618,#177619,#177620,#177621,#177622,#177623,
#177624,#177625,#177626,#177627,#177628),.UNSPECIFIED.,.F.,.F.,(4,3,3,3,
3,3,3,3,3,3,3,3,4),(0.,1.12535551670948E-5,7.76936938452495E-5,0.000102513517961045,
0.000121879189824203,0.000189659041345256,0.000223548967105782,0.000257294099096104,
0.000257438892866309,0.0003257208517583,0.000396486773960412,0.000466242707668339,
0.000514877785732617),.UNSPECIFIED.);
#4476=B_SPLINE_CURVE_WITH_KNOTS('',3,(#177636,#177637,#177638,#177639,#177640,
#177641,#177642,#177643,#177644,#177645,#177646,#177647,#177648,#177649,
#177650,#177651,#177652,#177653,#177654,#177655,#177656,#177657,#177658,
#177659,#177660,#177661,#177662,#177663,#177664,#177665,#177666,#177667,
#177668,#177669,#177670,#177671,#177672,#177673,#177674,#177675),
 .UNSPECIFIED.,.F.,.F.,(4,3,3,3,3,3,3,3,3,3,3,3,3,4),(0.,6.80370855368213E-5,
0.00013730316929917,0.000203636706664817,0.000256396220959701,0.000256540237295725,
0.000285209320207718,0.000342105100635639,0.00038477693595658,0.000400778874201932,
0.000456785658060667,0.000484789049990034,0.000498790745954718,0.000512792441919401),
 .UNSPECIFIED.);
#4477=B_SPLINE_CURVE_WITH_KNOTS('',3,(#177679,#177680,#177681,#177682,#177683,
#177684,#177685,#177686,#177687,#177688,#177689,#177690,#177691,#177692,
#177693,#177694,#177695,#177696,#177697,#177698,#177699,#177700,#177701,
#177702,#177703,#177704,#177705,#177706,#177707,#177708,#177709,#177710,
#177711,#177712,#177713,#177714,#177715),.UNSPECIFIED.,.F.,.F.,(4,3,3,3,
3,3,3,3,3,3,3,3,4),(0.,1.12535551670986E-5,7.76936938620434E-5,0.000102513517961113,
0.000121879189824263,0.000189659041345287,0.000223548967105799,0.000257294099096108,
0.000257438892866311,0.000325720851745853,0.000396486773936162,0.000466242707634991,
0.000514877785732623),.UNSPECIFIED.);
#4478=B_SPLINE_CURVE_WITH_KNOTS('',3,(#177723,#177724,#177725,#177726,#177727,
#177728,#177729,#177730,#177731,#177732,#177733,#177734,#177735,#177736,
#177737,#177738,#177739,#177740,#177741,#177742,#177743,#177744,#177745,
#177746,#177747,#177748,#177749,#177750,#177751,#177752,#177753,#177754,
#177755,#177756,#177757,#177758,#177759,#177760,#177761,#177762),
 .UNSPECIFIED.,.F.,.F.,(4,3,3,3,3,3,3,3,3,3,3,3,3,4),(0.,6.80370855419168E-5,
0.000137303169309447,0.000203636706680337,0.000256396220959704,0.000256540237295742,
0.000285209320207732,0.000342105100635651,0.00038477693595659,0.000400778874201942,
0.000456785658060675,0.000484789049990041,0.000498790745954724,0.000512792441919408),
 .UNSPECIFIED.);
#4479=B_SPLINE_CURVE_WITH_KNOTS('',3,(#177766,#177767,#177768,#177769,#177770,
#177771,#177772,#177773,#177774,#177775,#177776,#177777,#177778,#177779,
#177780,#177781,#177782,#177783,#177784,#177785,#177786,#177787,#177788,
#177789,#177790,#177791,#177792,#177793,#177794,#177795,#177796,#177797,
#177798,#177799,#177800,#177801,#177802),.UNSPECIFIED.,.F.,.F.,(4,3,3,3,
3,3,3,3,3,3,3,3,4),(0.,1.12535551670945E-5,7.76936938530435E-5,0.000102513517961046,
0.000121879189824204,0.000189659041345257,0.000223548967105783,0.0002572940990961,
0.000257438892866309,0.000325720851758386,0.000396486773961598,0.000466242707672009,
0.000514877785732619),.UNSPECIFIED.);
#4480=B_SPLINE_CURVE_WITH_KNOTS('',3,(#177810,#177811,#177812,#177813,#177814,
#177815,#177816,#177817,#177818,#177819,#177820,#177821,#177822,#177823,
#177824,#177825,#177826,#177827,#177828,#177829,#177830,#177831,#177832,
#177833,#177834,#177835,#177836,#177837,#177838,#177839,#177840,#177841,
#177842,#177843,#177844,#177845,#177846,#177847,#177848,#177849),
 .UNSPECIFIED.,.F.,.F.,(4,3,3,3,3,3,3,3,3,3,3,3,3,4),(0.,6.80370855335525E-5,
0.000137303169292306,0.000203636706653932,0.00025639622095971,0.000256540237295747,
0.000285209320207735,0.000342105100635656,0.000384776935956597,0.00040077887420195,
0.000456785658060685,0.000484789049990053,0.000498790745954737,0.00051279244191942),
 .UNSPECIFIED.);
#4481=B_SPLINE_CURVE_WITH_KNOTS('',3,(#177853,#177854,#177855,#177856,#177857,
#177858,#177859,#177860,#177861,#177862,#177863,#177864,#177865,#177866,
#177867,#177868,#177869,#177870,#177871,#177872,#177873,#177874,#177875,
#177876,#177877,#177878,#177879,#177880,#177881,#177882,#177883,#177884,
#177885,#177886,#177887,#177888,#177889),.UNSPECIFIED.,.F.,.F.,(4,3,3,3,
3,3,3,3,3,3,3,3,4),(0.,1.12535551670982E-5,7.76936938420302E-5,0.000102513517961121,
0.000121879189824269,0.000189659041345284,0.000223548967105792,0.00025729409909609,
0.000257438892866299,0.000325720851756146,0.000396486773955559,0.000466242707660611,
0.000514877785732599),.UNSPECIFIED.);
#4482=B_SPLINE_CURVE_WITH_KNOTS('',3,(#177897,#177898,#177899,#177900,#177901,
#177902,#177903,#177904,#177905,#177906,#177907,#177908,#177909,#177910,
#177911,#177912,#177913,#177914,#177915,#177916,#177917,#177918,#177919,
#177920,#177921,#177922,#177923,#177924,#177925,#177926,#177927,#177928,
#177929,#177930,#177931,#177932,#177933,#177934,#177935,#177936),
 .UNSPECIFIED.,.F.,.F.,(4,3,3,3,3,3,3,3,3,3,3,3,3,4),(0.,6.80370855388716E-5,
0.000137303169302875,0.00020363670666931,0.000256396220959701,0.000256540237295736,
0.000285209320207724,0.000342105100635644,0.000384776935956583,0.000400778874201936,
0.000456785658060669,0.000484789049990036,0.000498790745954719,0.000512792441919403),
 .UNSPECIFIED.);
#4483=B_SPLINE_CURVE_WITH_KNOTS('',3,(#177940,#177941,#177942,#177943,#177944,
#177945,#177946,#177947,#177948,#177949,#177950,#177951,#177952,#177953,
#177954,#177955,#177956,#177957,#177958,#177959,#177960,#177961,#177962,
#177963,#177964,#177965,#177966,#177967,#177968,#177969,#177970,#177971,
#177972,#177973,#177974,#177975,#177976),.UNSPECIFIED.,.F.,.F.,(4,3,3,3,
3,3,3,3,3,3,3,3,4),(0.,1.12535551670968E-5,7.76936938432487E-5,0.000102513517961121,
0.000121879189824269,0.000189659041345286,0.000223548967105795,0.000257294099096113,
0.000257438892866304,0.000325720851757511,0.000396486773960315,0.000466242707671397,
0.000514877785732607),.UNSPECIFIED.);
#4484=B_SPLINE_CURVE_WITH_KNOTS('',3,(#177984,#177985,#177986,#177987,#177988,
#177989,#177990,#177991,#177992,#177993,#177994,#177995,#177996,#177997,
#177998,#177999,#178000,#178001,#178002,#178003,#178004,#178005,#178006,
#178007,#178008,#178009,#178010,#178011,#178012,#178013,#178014,#178015,
#178016,#178017,#178018,#178019,#178020,#178021,#178022,#178023),
 .UNSPECIFIED.,.F.,.F.,(4,3,3,3,3,3,3,3,3,3,3,3,3,4),(0.,6.80370855309538E-5,
0.00013730316928727,0.000203636706647231,0.000256396220959712,0.000256540237295743,
0.000285209320207748,0.000342105100635667,0.000384776935956606,0.000400778874201958,
0.000456785658060691,0.000484789049990057,0.000498790745954741,0.000512792441919424),
 .UNSPECIFIED.);
#4485=B_SPLINE_CURVE_WITH_KNOTS('',3,(#178027,#178028,#178029,#178030,#178031,
#178032,#178033,#178034,#178035,#178036,#178037,#178038,#178039,#178040,
#178041,#178042,#178043,#178044,#178045,#178046,#178047,#178048,#178049,
#178050,#178051,#178052,#178053,#178054,#178055,#178056,#178057,#178058,
#178059,#178060,#178061,#178062,#178063),.UNSPECIFIED.,.F.,.F.,(4,3,3,3,
3,3,3,3,3,3,3,3,4),(0.,1.12535551670983E-5,7.76936938367873E-5,0.000102513517961129,
0.000121879189824276,0.000189659041345291,0.000223548967105798,0.000257294099096089,
0.000257438892866305,0.000325720851750639,0.000396486773945176,0.000466242707647004,
0.00051487778573261),.UNSPECIFIED.);
#4486=B_SPLINE_CURVE_WITH_KNOTS('',3,(#178071,#178072,#178073,#178074,#178075,
#178076,#178077,#178078,#178079,#178080,#178081,#178082,#178083,#178084,
#178085,#178086,#178087,#178088,#178089,#178090,#178091,#178092,#178093,
#178094,#178095,#178096,#178097,#178098,#178099,#178100,#178101,#178102,
#178103,#178104,#178105,#178106,#178107,#178108,#178109,#178110),
 .UNSPECIFIED.,.F.,.F.,(4,3,3,3,3,3,3,3,3,3,3,3,3,4),(0.,6.80370855382641E-5,
0.000137303169301827,0.000203636706668335,0.000256396220959708,0.000256540237295738,
0.000285209320207749,0.000342105100635665,0.000384776935956603,0.000400778874201954,
0.000456785658060685,0.00048478904999005,0.000498790745954732,0.000512792441919415),
 .UNSPECIFIED.);
#4487=B_SPLINE_CURVE_WITH_KNOTS('',3,(#178114,#178115,#178116,#178117,#178118,
#178119,#178120,#178121,#178122,#178123,#178124,#178125,#178126,#178127,
#178128,#178129,#178130,#178131,#178132,#178133,#178134,#178135,#178136,
#178137,#178138,#178139,#178140,#178141,#178142,#178143,#178144,#178145,
#178146,#178147,#178148,#178149,#178150),.UNSPECIFIED.,.F.,.F.,(4,3,3,3,
3,3,3,3,3,3,3,3,4),(0.,1.12535551670954E-5,7.769369383202E-5,0.000102513517961085,
0.000121879189824237,0.00018965904134527,0.000223548967105787,0.000257294099096099,
0.000257438892866304,0.000325720851760152,0.000396486773964489,0.000466242707675398,
0.000514877785732607),.UNSPECIFIED.);
#4488=B_SPLINE_CURVE_WITH_KNOTS('',3,(#178158,#178159,#178160,#178161,#178162,
#178163,#178164,#178165,#178166,#178167,#178168,#178169,#178170,#178171,
#178172,#178173,#178174,#178175,#178176,#178177,#178178,#178179,#178180,
#178181,#178182,#178183,#178184,#178185,#178186,#178187,#178188,#178189,
#178190,#178191,#178192,#178193,#178194,#178195,#178196,#178197),
 .UNSPECIFIED.,.F.,.F.,(4,3,3,3,3,3,3,3,3,3,3,3,3,4),(0.,6.80370855357845E-5,
0.000137303169296545,0.000203636706659477,0.000256396220959712,0.000256540237295743,
0.000285209320207756,0.000342105100635673,0.000384776935956611,0.000400778874201962,
0.000456785658060693,0.000484789049990058,0.000498790745954741,0.000512792441919424),
 .UNSPECIFIED.);
#4489=B_SPLINE_CURVE_WITH_KNOTS('',3,(#178201,#178202,#178203,#178204,#178205,
#178206,#178207,#178208,#178209,#178210,#178211,#178212,#178213,#178214,
#178215,#178216,#178217,#178218,#178219,#178220,#178221,#178222,#178223,
#178224,#178225,#178226,#178227,#178228,#178229,#178230,#178231,#178232,
#178233,#178234,#178235,#178236,#178237),.UNSPECIFIED.,.F.,.F.,(4,3,3,3,
3,3,3,3,3,3,3,3,4),(0.,1.12535551670973E-5,7.76936938384776E-5,0.000102513517961114,
0.000121879189824263,0.000189659041345285,0.000223548967105795,0.000257294099096104,
0.000257438892866306,0.000325720851762052,0.000396486773967539,0.000466242707677798,
0.000514877785732612),.UNSPECIFIED.);
#4490=B_SPLINE_CURVE_WITH_KNOTS('',3,(#178245,#178246,#178247,#178248,#178249,
#178250,#178251,#178252,#178253,#178254,#178255,#178256,#178257,#178258,
#178259,#178260,#178261,#178262,#178263,#178264,#178265,#178266,#178267,
#178268,#178269,#178270,#178271,#178272,#178273,#178274,#178275,#178276,
#178277,#178278,#178279,#178280,#178281,#178282,#178283,#178284),
 .UNSPECIFIED.,.F.,.F.,(4,3,3,3,3,3,3,3,3,3,3,3,3,4),(0.,6.80370855448908E-5,
0.00013730316931562,0.000203636706689471,0.000256396220959709,0.000256540237295741,
0.000285209320207744,0.000342105100635662,0.000384776935956601,0.000400778874201953,
0.000456785658060685,0.000484789049990051,0.000498790745954734,0.000512792441919417),
 .UNSPECIFIED.);
#4491=B_SPLINE_CURVE_WITH_KNOTS('',3,(#178288,#178289,#178290,#178291,#178292,
#178293,#178294,#178295,#178296,#178297,#178298,#178299,#178300,#178301,
#178302,#178303,#178304,#178305,#178306,#178307,#178308,#178309,#178310,
#178311,#178312,#178313,#178314,#178315,#178316,#178317,#178318,#178319,
#178320,#178321,#178322,#178323,#178324),.UNSPECIFIED.,.F.,.F.,(4,3,3,3,
3,3,3,3,3,3,3,3,4),(0.,1.12535551670965E-5,7.7693693850504E-5,0.000102513517961145,
0.00012187918982429,0.000189659041345294,0.000223548967105797,0.000257294099096094,
0.000257438892866299,0.000325720851758731,0.000396486773961765,0.000466242707671255,
0.000514877785732599),.UNSPECIFIED.);
#4492=B_SPLINE_CURVE_WITH_KNOTS('',3,(#178332,#178333,#178334,#178335,#178336,
#178337,#178338,#178339,#178340,#178341,#178342,#178343,#178344,#178345,
#178346,#178347,#178348,#178349,#178350,#178351,#178352,#178353,#178354,
#178355,#178356,#178357,#178358,#178359,#178360,#178361,#178362,#178363,
#178364,#178365,#178366,#178367,#178368,#178369,#178370,#178371),
 .UNSPECIFIED.,.F.,.F.,(4,3,3,3,3,3,3,3,3,3,3,3,3,4),(0.,6.80370855381794E-5,
0.000137303169301656,0.000203636706667918,0.000256396220959708,0.000256540237295746,
0.000285209320207746,0.000342105100635663,0.000384776935956602,0.000400778874201954,
0.000456785658060685,0.000484789049990051,0.000498790745954734,0.000512792441919417),
 .UNSPECIFIED.);
#4493=B_SPLINE_CURVE_WITH_KNOTS('',3,(#178375,#178376,#178377,#178378,#178379,
#178380,#178381,#178382,#178383,#178384,#178385,#178386,#178387,#178388,
#178389,#178390,#178391,#178392,#178393,#178394,#178395,#178396,#178397,
#178398,#178399,#178400,#178401,#178402,#178403,#178404,#178405,#178406,
#178407,#178408,#178409,#178410,#178411),.UNSPECIFIED.,.F.,.F.,(4,3,3,3,
3,3,3,3,3,3,3,3,4),(0.,1.12535551670961E-5,7.76936938492663E-5,0.000102513517961084,
0.000121879189824237,0.00018965904134527,0.000223548967105786,0.000257294099096085,
0.000257438892866303,0.000325720851754593,0.00039648677395353,0.000466242707659808,
0.000514877785732606),.UNSPECIFIED.);
#4494=B_SPLINE_CURVE_WITH_KNOTS('',3,(#178418,#178419,#178420,#178421,#178422,
#178423,#178424,#178425,#178426,#178427,#178428,#178429,#178430,#178431,
#178432,#178433,#178434,#178435,#178436,#178437,#178438,#178439,#178440,
#178441,#178442,#178443,#178444,#178445,#178446,#178447,#178448,#178449,
#178450,#178451,#178452,#178453,#178454,#178455,#178456,#178457),
 .UNSPECIFIED.,.F.,.F.,(4,3,3,3,3,3,3,3,3,3,3,3,3,4),(0.,6.80370855321557E-5,
0.000137303169289422,0.000203636706649785,0.000256396220959709,0.000256540237295743,
0.000285209320207743,0.000342105100635662,0.000384776935956601,0.000400778874201953,
0.000456785658060685,0.000484789049990051,0.000498790745954734,0.000512792441919417),
 .UNSPECIFIED.);
#4495=B_SPLINE_CURVE_WITH_KNOTS('',3,(#182071,#182072,#182073,#182074,#182075,
#182076,#182077,#182078,#182079,#182080,#182081,#182082,#182083,#182084,
#182085,#182086,#182087,#182088,#182089,#182090,#182091,#182092,#182093,
#182094,#182095,#182096,#182097,#182098,#182099,#182100,#182101,#182102,
#182103,#182104,#182105,#182106,#182107,#182108,#182109,#182110,#182111,
#182112,#182113,#182114,#182115,#182116,#182117,#182118,#182119,#182120,
#182121,#182122),.UNSPECIFIED.,.F.,.F.,(4,3,3,3,3,3,3,3,3,3,3,3,3,3,3,3,
3,4),(0.,4.3070623787495E-5,8.47417087705792E-5,0.000124159989206991,0.000160467076291534,
0.0001709983821167,0.000182414994733782,0.000213747977645871,0.000242415955902806,
0.000256497573175043,0.000259169422895616,0.000261757777312422,0.000289965130403398,
0.000301877270772904,0.000321937017503146,0.000326951954185706,0.000334474359209546,
0.000341996764233387),.UNSPECIFIED.);
#4496=B_SPLINE_CURVE_WITH_KNOTS('',3,(#182123,#182124,#182125,#182126,#182127,
#182128,#182129,#182130,#182131,#182132,#182133,#182134,#182135,#182136,
#182137,#182138,#182139,#182140,#182141,#182142,#182143,#182144,#182145,
#182146,#182147,#182148,#182149,#182150,#182151,#182152,#182153,#182154,
#182155,#182156,#182157,#182158,#182159,#182160,#182161,#182162,#182163,
#182164,#182165,#182166,#182167,#182168,#182169,#182170,#182171,#182172,
#182173,#182174),.UNSPECIFIED.,.F.,.F.,(4,3,3,3,3,3,3,3,3,3,3,3,3,3,3,3,
3,4),(0.,2.58457451675486E-5,4.25394446196056E-5,6.4665986968724E-5,7.57292581432831E-5,
8.12608937305627E-5,8.26438026273826E-5,8.67925293178423E-5,0.000116015624428002,
0.000130188793976763,0.000151886926306224,0.00016196365121129,0.000162735992470954,
0.000173585058635685,0.000212487880460513,0.000255238173511739,0.000301397761149341,
0.000347170117271356),.UNSPECIFIED.);
#4497=B_SPLINE_CURVE_WITH_KNOTS('',3,(#182176,#182177,#182178,#182179,#182180,
#182181,#182182,#182183,#182184,#182185,#182186,#182187,#182188,#182189,
#182190,#182191,#182192,#182193,#182194,#182195,#182196,#182197,#182198,
#182199,#182200,#182201,#182202,#182203,#182204,#182205,#182206,#182207,
#182208,#182209,#182210,#182211,#182212,#182213,#182214,#182215,#182216,
#182217,#182218,#182219,#182220,#182221),.UNSPECIFIED.,.F.,.F.,(4,3,3,3,
3,3,3,3,3,3,3,3,3,3,3,4),(3.3881317890172E-21,2.57218161986703E-5,4.21568322567895E-5,
6.4587331461705E-5,7.58025810641627E-5,8.14102058653916E-5,8.28121120656988E-5,
8.70178306666205E-5,0.000116081955657568,0.000130526745999931,0.00016239411102205,
0.000174035661333241,0.000213138396956876,0.000256116935431032,0.000302406662851701,
0.000348071322666469),.UNSPECIFIED.);
#4498=B_SPLINE_CURVE_WITH_KNOTS('',3,(#182222,#182223,#182224,#182225,#182226,
#182227,#182228,#182229,#182230,#182231,#182232,#182233,#182234,#182235,
#182236,#182237,#182238,#182239,#182240,#182241,#182242,#182243,#182244,
#182245,#182246,#182247,#182248,#182249,#182250,#182251,#182252,#182253,
#182254,#182255,#182256,#182257,#182258,#182259,#182260,#182261,#182262,
#182263,#182264,#182265,#182266,#182267,#182268,#182269,#182270,#182271,
#182272,#182273),.UNSPECIFIED.,.F.,.F.,(4,3,3,3,3,3,3,3,3,3,3,3,3,3,3,3,
3,4),(0.,4.29652152163274E-5,8.4451910753757E-5,0.000123669830865422,0.000159788877358504,
0.000170558847912626,0.000181218775907166,0.000181960046452408,0.000214460062643432,
0.000244755726198055,0.000255838271868945,0.00025850325386758,0.000261084955178757,
0.000289370476647835,0.000301101325502011,0.000321109510663637,0.000331113603244451,
0.000341117695825264),.UNSPECIFIED.);
#4499=B_SPLINE_CURVE_WITH_KNOTS('',3,(#185956,#185957,#185958,#185959,#185960,
#185961,#185962,#185963,#185964,#185965,#185966,#185967,#185968,#185969,
#185970,#185971,#185972,#185973,#185974,#185975,#185976,#185977,#185978,
#185979,#185980,#185981,#185982,#185983,#185984,#185985,#185986,#185987,
#185988,#185989,#185990,#185991,#185992,#185993,#185994,#185995,#185996,
#185997,#185998,#185999,#186000,#186001,#186002,#186003,#186004,#186005,
#186006,#186007),.UNSPECIFIED.,.F.,.F.,(4,3,3,3,3,3,3,3,3,3,3,3,3,3,3,3,
3,4),(0.,4.30706237904622E-5,8.47417087758447E-5,0.000124159989214271,0.000160467076301093,
0.00017099838211669,0.000182414994733772,0.000213747977645865,0.000242415955903934,
0.00025649757317504,0.000259169422895614,0.000261757777312419,0.000289965130401458,
0.000301877270772905,0.000321937017503148,0.000326951954185709,0.00033447435920955,
0.000341996764233391),.UNSPECIFIED.);
#4500=B_SPLINE_CURVE_WITH_KNOTS('',3,(#186008,#186009,#186010,#186011,#186012,
#186013,#186014,#186015,#186016,#186017,#186018,#186019,#186020,#186021,
#186022,#186023,#186024,#186025,#186026,#186027,#186028,#186029,#186030,
#186031,#186032,#186033,#186034,#186035,#186036,#186037,#186038,#186039,
#186040,#186041,#186042,#186043,#186044,#186045,#186046,#186047,#186048,
#186049,#186050,#186051,#186052,#186053,#186054,#186055,#186056,#186057,
#186058,#186059),.UNSPECIFIED.,.F.,.F.,(4,3,3,3,3,3,3,3,3,3,3,3,3,3,3,3,
3,4),(8.67361737988404E-19,2.58457451683905E-5,4.25394446195019E-5,6.4665986968671E-5,
7.57292581432556E-5,8.12608937305479E-5,8.26438026273709E-5,8.67925293178401E-5,
0.000116015624426893,0.00013018879397676,0.00015188692630622,0.000161963651211285,
0.00016273599247095,0.000173585058635679,0.000212487880462509,0.000255238173515559,
0.000301397761155017,0.000347170117271358),.UNSPECIFIED.);
#4501=B_SPLINE_CURVE_WITH_KNOTS('',3,(#186061,#186062,#186063,#186064,#186065,
#186066,#186067,#186068,#186069,#186070,#186071,#186072,#186073,#186074,
#186075,#186076,#186077,#186078,#186079,#186080,#186081,#186082,#186083,
#186084,#186085,#186086,#186087,#186088,#186089,#186090,#186091,#186092,
#186093,#186094,#186095,#186096,#186097,#186098,#186099,#186100,#186101,
#186102,#186103,#186104,#186105,#186106),.UNSPECIFIED.,.F.,.F.,(4,3,3,3,
3,3,3,3,3,3,3,3,3,3,3,4),(0.,2.57218162004654E-5,4.21568322569402E-5,6.4587331461781E-5,
7.58025810642015E-5,8.14102058654117E-5,8.28121120657143E-5,8.7017830666622E-5,
0.000116081955658923,0.000130526745999929,0.000162394111022053,0.000174035661333236,
0.000213138396959096,0.000256116935435479,0.000302406662858657,0.000348071322666466),
 .UNSPECIFIED.);
#4502=B_SPLINE_CURVE_WITH_KNOTS('',3,(#186107,#186108,#186109,#186110,#186111,
#186112,#186113,#186114,#186115,#186116,#186117,#186118,#186119,#186120,
#186121,#186122,#186123,#186124,#186125,#186126,#186127,#186128,#186129,
#186130,#186131,#186132,#186133,#186134,#186135,#186136,#186137,#186138,
#186139,#186140,#186141,#186142,#186143,#186144,#186145,#186146,#186147,
#186148,#186149,#186150,#186151,#186152,#186153,#186154,#186155,#186156,
#186157,#186158),.UNSPECIFIED.,.F.,.F.,(4,3,3,3,3,3,3,3,3,3,3,3,3,3,3,3,
3,4),(0.,4.29652152126473E-5,8.44519107477571E-5,0.000123669830857838,0.000159788877349733,
0.000170558847912618,0.000181218775907158,0.000181960046452388,0.000214460062643972,
0.000244755726199678,0.00025583827186894,0.000258503253867575,0.000261084955178752,
0.000289370476647328,0.000301101325502007,0.000321109510663634,0.000331113603244448,
0.000341117695825262),.UNSPECIFIED.);
#4503=B_SPLINE_CURVE_WITH_KNOTS('',3,(#186160,#186161,#186162,#186163,#186164,
#186165,#186166,#186167,#186168,#186169,#186170,#186171,#186172,#186173,
#186174,#186175,#186176,#186177,#186178,#186179,#186180,#186181,#186182,
#186183,#186184,#186185,#186186,#186187,#186188,#186189,#186190,#186191,
#186192,#186193,#186194,#186195,#186196,#186197,#186198,#186199,#186200,
#186201,#186202,#186203,#186204,#186205,#186206,#186207,#186208,#186209,
#186210,#186211),.UNSPECIFIED.,.F.,.F.,(4,3,3,3,3,3,3,3,3,3,3,3,3,3,3,3,
3,4),(0.,4.30706237869498E-5,8.47417087696762E-5,0.000124159989205771,0.000160467076290074,
0.000170998382116688,0.000182414994733765,0.000213747977645863,0.000242415955902775,
0.000256497573175039,0.000259169422895612,0.000261757777312418,0.000289965130403254,
0.000301877270772904,0.000321937017503147,0.000326951954185708,0.000334474359209549,
0.00034199676423339),.UNSPECIFIED.);
#4504=B_SPLINE_CURVE_WITH_KNOTS('',3,(#186212,#186213,#186214,#186215,#186216,
#186217,#186218,#186219,#186220,#186221,#186222,#186223,#186224,#186225,
#186226,#186227,#186228,#186229,#186230,#186231,#186232,#186233,#186234,
#186235,#186236,#186237,#186238,#186239,#186240,#186241,#186242,#186243,
#186244,#186245,#186246,#186247,#186248,#186249,#186250,#186251,#186252,
#186253,#186254,#186255,#186256,#186257,#186258,#186259,#186260,#186261,
#186262,#186263),.UNSPECIFIED.,.F.,.F.,(4,3,3,3,3,3,3,3,3,3,3,3,3,3,3,3,
3,4),(0.,2.58457451680011E-5,4.25394446195326E-5,6.46659869686882E-5,7.5729258143266E-5,
8.12608937305549E-5,8.26438026273771E-5,8.67925293178438E-5,0.000116015624426372,
0.000130188793976766,0.000151886926306227,0.000161963651211297,0.000162735992470957,
0.000173585058635688,0.000212487880459008,0.000255238173508161,0.00030139776114258,
0.000347170117271372),.UNSPECIFIED.);
#4505=B_SPLINE_CURVE_WITH_KNOTS('',3,(#186265,#186266,#186267,#186268,#186269,
#186270,#186271,#186272,#186273,#186274,#186275,#186276,#186277,#186278,
#186279,#186280,#186281,#186282,#186283,#186284,#186285,#186286,#186287,
#186288,#186289,#186290,#186291,#186292,#186293,#186294,#186295,#186296,
#186297,#186298,#186299,#186300,#186301,#186302,#186303,#186304,#186305,
#186306,#186307,#186308,#186309,#186310),.UNSPECIFIED.,.F.,.F.,(4,3,3,3,
3,3,3,3,3,3,3,3,3,3,3,4),(1.73472347597681E-18,2.57218161995936E-5,4.21568322567643E-5,
6.45873314616834E-5,7.5802581064143E-5,8.14102058653728E-5,8.28121120656802E-5,
8.70178306666025E-5,0.000116081955658033,0.000130526745999903,0.000162394111022011,
0.000174035661333203,0.000213138396957744,0.000256116935432899,0.000302406662854991,
0.000348071322666432),.UNSPECIFIED.);
#4506=B_SPLINE_CURVE_WITH_KNOTS('',3,(#186311,#186312,#186313,#186314,#186315,
#186316,#186317,#186318,#186319,#186320,#186321,#186322,#186323,#186324,
#186325,#186326,#186327,#186328,#186329,#186330,#186331,#186332,#186333,
#186334,#186335,#186336,#186337,#186338,#186339,#186340,#186341,#186342,
#186343,#186344,#186345,#186346,#186347,#186348,#186349,#186350,#186351,
#186352,#186353,#186354,#186355,#186356,#186357,#186358,#186359,#186360,
#186361,#186362),.UNSPECIFIED.,.F.,.F.,(4,3,3,3,3,3,3,3,3,3,3,3,3,3,3,3,
3,4),(0.,4.2965215218261E-5,8.44519107571648E-5,0.00012366983086999,0.000159788877364278,
0.000170558847912618,0.000181218775907157,0.000181960046452381,0.000214460062644312,
0.000244755726200678,0.000255838271868933,0.000258503253867568,0.000261084955178745,
0.000289370476645579,0.000301101325501997,0.000321109510663622,0.000331113603244435,
0.000341117695825248),.UNSPECIFIED.);
#4507=B_SPLINE_CURVE_WITH_KNOTS('',3,(#186364,#186365,#186366,#186367,#186368,
#186369,#186370,#186371,#186372,#186373,#186374,#186375,#186376,#186377,
#186378,#186379,#186380,#186381,#186382,#186383,#186384,#186385,#186386,
#186387,#186388,#186389,#186390,#186391,#186392,#186393,#186394,#186395,
#186396,#186397,#186398,#186399,#186400,#186401,#186402,#186403,#186404,
#186405,#186406,#186407,#186408,#186409,#186410,#186411,#186412,#186413,
#186414,#186415),.UNSPECIFIED.,.F.,.F.,(4,3,3,3,3,3,3,3,3,3,3,3,3,3,3,3,
3,4),(9.81307786677359E-18,4.30706237872886E-5,8.47417087703267E-5,0.000124159989206749,
0.000160467076291443,0.000170998382116702,0.000182414994733785,0.000213747977645874,
0.000242415955904002,0.000256497573175045,0.000259169422895618,0.000261757777312424,
0.000289965130402902,0.000301877270772906,0.000321937017503147,0.000326951954185707,
0.000334474359209548,0.000341996764233388),.UNSPECIFIED.);
#4508=B_SPLINE_CURVE_WITH_KNOTS('',3,(#186416,#186417,#186418,#186419,#186420,
#186421,#186422,#186423,#186424,#186425,#186426,#186427,#186428,#186429,
#186430,#186431,#186432,#186433,#186434,#186435,#186436,#186437,#186438,
#186439,#186440,#186441,#186442,#186443,#186444,#186445,#186446,#186447,
#186448,#186449,#186450,#186451,#186452,#186453,#186454,#186455,#186456,
#186457,#186458,#186459,#186460,#186461,#186462,#186463,#186464,#186465,
#186466,#186467),.UNSPECIFIED.,.F.,.F.,(4,3,3,3,3,3,3,3,3,3,3,3,3,3,3,3,
3,4),(0.,2.58457451681907E-5,4.25394446194808E-5,6.46659869686619E-5,7.57292581432524E-5,
8.12608937305477E-5,8.26438026273715E-5,8.67925293178429E-5,0.000116015624427697,
0.000130188793976764,0.000151886926306225,0.000161963651211284,0.000162735992470955,
0.000173585058635686,0.000212487880460992,0.000255238173511379,0.000301397761145688,
0.000347170117271377),.UNSPECIFIED.);
#4509=B_SPLINE_CURVE_WITH_KNOTS('',3,(#186469,#186470,#186471,#186472,#186473,
#186474,#186475,#186476,#186477,#186478,#186479,#186480,#186481,#186482,
#186483,#186484,#186485,#186486,#186487,#186488,#186489,#186490,#186491,
#186492,#186493,#186494,#186495,#186496,#186497,#186498,#186499,#186500,
#186501,#186502,#186503,#186504,#186505,#186506,#186507,#186508,#186509,
#186510,#186511,#186512,#186513,#186514),.UNSPECIFIED.,.F.,.F.,(4,3,3,3,
3,3,3,3,3,3,3,3,3,3,3,4),(0.,2.57218161996713E-5,4.2156832256742E-5,6.45873314616798E-5,
7.58025810641487E-5,8.14102058653831E-5,8.28121120656917E-5,8.70178306666176E-5,
0.000116081955658986,0.000130526745999926,0.000162394111022057,0.000174035661333235,
0.000213138396960236,0.000256116935437692,0.000302406662861853,0.000348071322666466),
 .UNSPECIFIED.);
#4510=B_SPLINE_CURVE_WITH_KNOTS('',3,(#186515,#186516,#186517,#186518,#186519,
#186520,#186521,#186522,#186523,#186524,#186525,#186526,#186527,#186528,
#186529,#186530,#186531,#186532,#186533,#186534,#186535,#186536,#186537,
#186538,#186539,#186540,#186541,#186542,#186543,#186544,#186545,#186546,
#186547,#186548,#186549,#186550,#186551,#186552,#186553,#186554,#186555,
#186556,#186557,#186558,#186559,#186560,#186561,#186562,#186563,#186564,
#186565,#186566),.UNSPECIFIED.,.F.,.F.,(4,3,3,3,3,3,3,3,3,3,3,3,3,3,3,3,
3,4),(0.,4.29652152153032E-5,8.44519107518936E-5,0.000123669830862718,0.000159788877354853,
0.000170558847912617,0.000181218775907157,0.000181960046452383,0.000214460062643983,
0.000244755726199726,0.00025583827186894,0.000258503253867575,0.000261084955178752,
0.000289370476647621,0.000301101325502007,0.000321109510663635,0.000331113603244448,
0.000341117695825262),.UNSPECIFIED.);
#4511=B_SPLINE_CURVE_WITH_KNOTS('',3,(#186568,#186569,#186570,#186571,#186572,
#186573,#186574,#186575,#186576,#186577,#186578,#186579,#186580,#186581,
#186582,#186583,#186584,#186585,#186586,#186587,#186588,#186589,#186590,
#186591,#186592,#186593,#186594,#186595,#186596,#186597,#186598,#186599,
#186600,#186601,#186602,#186603,#186604,#186605,#186606,#186607,#186608,
#186609,#186610,#186611,#186612,#186613,#186614,#186615,#186616,#186617,
#186618,#186619),.UNSPECIFIED.,.F.,.F.,(4,3,3,3,3,3,3,3,3,3,3,3,3,3,3,3,
3,4),(0.,4.30706237883116E-5,8.4741708772137E-5,0.000124159989209315,0.000160467076294801,
0.000170998382116688,0.000182414994733781,0.000213747977645863,0.000242415955903352,
0.000256497573175038,0.000259169422895611,0.000261757777312417,0.000289965130402052,
0.000301877270772902,0.000321937017503145,0.000326951954185706,0.000334474359209547,
0.000341996764233388),.UNSPECIFIED.);
#4512=B_SPLINE_CURVE_WITH_KNOTS('',3,(#186620,#186621,#186622,#186623,#186624,
#186625,#186626,#186627,#186628,#186629,#186630,#186631,#186632,#186633,
#186634,#186635,#186636,#186637,#186638,#186639,#186640,#186641,#186642,
#186643,#186644,#186645,#186646,#186647,#186648,#186649,#186650,#186651,
#186652,#186653,#186654,#186655,#186656,#186657,#186658,#186659,#186660,
#186661,#186662,#186663,#186664,#186665,#186666,#186667,#186668,#186669,
#186670,#186671),.UNSPECIFIED.,.F.,.F.,(4,3,3,3,3,3,3,3,3,3,3,3,3,3,3,3,
3,4),(0.,2.58457451672917E-5,4.25394446196108E-5,6.46659869687248E-5,7.57292581432817E-5,
8.12608937305602E-5,8.26438026273798E-5,8.67925293178387E-5,0.000116015624427758,
0.000130188793976758,0.000151886926306218,0.000161963651211268,0.000162735992470948,
0.000173585058635677,0.000212487880459398,0.00025523817350879,0.000301397761142968,
0.000347170117271355),.UNSPECIFIED.);
#4513=B_SPLINE_CURVE_WITH_KNOTS('',3,(#186673,#186674,#186675,#186676,#186677,
#186678,#186679,#186680,#186681,#186682,#186683,#186684,#186685,#186686,
#186687,#186688,#186689,#186690,#186691,#186692,#186693,#186694,#186695,
#186696,#186697,#186698,#186699,#186700,#186701,#186702,#186703,#186704,
#186705,#186706,#186707,#186708,#186709,#186710,#186711,#186712,#186713,
#186714,#186715,#186716,#186717,#186718),.UNSPECIFIED.,.F.,.F.,(4,3,3,3,
3,3,3,3,3,3,3,3,3,3,3,4),(3.46944695195361E-18,2.57218161983717E-5,4.21568322568919E-5,
6.45873314617591E-5,7.58025810641928E-5,8.14102058654096E-5,8.28121120657138E-5,
8.70178306666264E-5,0.000116081955657765,0.000130526745999938,0.000162394111022065,
0.000174035661333249,0.000213138396958737,0.000256116935434866,0.000302406662858167,
0.000348071322666474),.UNSPECIFIED.);
#4514=B_SPLINE_CURVE_WITH_KNOTS('',3,(#186719,#186720,#186721,#186722,#186723,
#186724,#186725,#186726,#186727,#186728,#186729,#186730,#186731,#186732,
#186733,#186734,#186735,#186736,#186737,#186738,#186739,#186740,#186741,
#186742,#186743,#186744,#186745,#186746,#186747,#186748,#186749,#186750,
#186751,#186752,#186753,#186754,#186755,#186756,#186757,#186758,#186759,
#186760,#186761,#186762,#186763,#186764,#186765,#186766,#186767,#186768,
#186769,#186770),.UNSPECIFIED.,.F.,.F.,(4,3,3,3,3,3,3,3,3,3,3,3,3,3,3,3,
3,4),(0.,4.29652152163865E-5,8.4451910753883E-5,0.000123669830865533,0.000159788877358621,
0.000170558847912619,0.000181218775907159,0.000181960046452386,0.000214460062643117,
0.000244755726196957,0.000255838271868941,0.000258503253867576,0.000261084955178754,
0.000289370476648858,0.000301101325502009,0.000321109510663636,0.00033111360324445,
0.000341117695825264),.UNSPECIFIED.);
#4515=B_SPLINE_CURVE_WITH_KNOTS('',3,(#186772,#186773,#186774,#186775,#186776,
#186777,#186778,#186779,#186780,#186781,#186782,#186783,#186784,#186785,
#186786,#186787,#186788,#186789,#186790,#186791,#186792,#186793,#186794,
#186795,#186796,#186797,#186798,#186799,#186800,#186801,#186802,#186803,
#186804,#186805,#186806,#186807,#186808,#186809,#186810,#186811,#186812,
#186813,#186814,#186815,#186816,#186817,#186818,#186819,#186820,#186821,
#186822,#186823),.UNSPECIFIED.,.F.,.F.,(4,3,3,3,3,3,3,3,3,3,3,3,3,3,3,3,
3,4),(0.,4.30706237866878E-5,8.47417087690751E-5,0.000124159989204751,0.000160467076288489,
0.000170998382116703,0.000182414994733785,0.000213747977645875,0.000242415955903625,
0.000256497573175048,0.000259169422895621,0.000261757777312427,0.000289965130402839,
0.00030187727077291,0.000321937017503152,0.000326951954185712,0.000334474359209553,
0.000341996764233393),.UNSPECIFIED.);
#4516=B_SPLINE_CURVE_WITH_KNOTS('',3,(#186824,#186825,#186826,#186827,#186828,
#186829,#186830,#186831,#186832,#186833,#186834,#186835,#186836,#186837,
#186838,#186839,#186840,#186841,#186842,#186843,#186844,#186845,#186846,
#186847,#186848,#186849,#186850,#186851,#186852,#186853,#186854,#186855,
#186856,#186857,#186858,#186859,#186860,#186861,#186862,#186863,#186864,
#186865,#186866,#186867,#186868,#186869,#186870,#186871,#186872,#186873,
#186874,#186875),.UNSPECIFIED.,.F.,.F.,(4,3,3,3,3,3,3,3,3,3,3,3,3,3,3,3,
3,4),(3.46944695195361E-18,2.58457451665415E-5,4.25394446196409E-5,6.4665986968742E-5,
7.57292581432925E-5,8.12608937305678E-5,8.26438026273866E-5,8.67925293178431E-5,
0.000116015624427815,0.000130188793976763,0.000151886926306223,0.000161963651211269,
0.000162735992470953,0.000173585058635683,0.000212487880462884,0.000255238173515455,
0.000301397761152582,0.000347170117271373),.UNSPECIFIED.);
#4517=B_SPLINE_CURVE_WITH_KNOTS('',3,(#186877,#186878,#186879,#186880,#186881,
#186882,#186883,#186884,#186885,#186886,#186887,#186888,#186889,#186890,
#186891,#186892,#186893,#186894,#186895,#186896,#186897,#186898,#186899,
#186900,#186901,#186902,#186903,#186904,#186905,#186906,#186907,#186908,
#186909,#186910,#186911,#186912,#186913,#186914,#186915,#186916,#186917,
#186918,#186919,#186920,#186921,#186922),.UNSPECIFIED.,.F.,.F.,(4,3,3,3,
3,3,3,3,3,3,3,3,3,3,3,4),(0.,2.57218162001907E-5,4.21568322567731E-5,6.45873314616956E-5,
7.58025810641568E-5,8.14102058653875E-5,8.28121120656951E-5,8.70178306666181E-5,
0.000116081955658954,0.000130526745999927,0.000162394111022066,0.000174035661333236,
0.000213138396957247,0.000256116935431918,0.000302406662853574,0.00034807132266646),
 .UNSPECIFIED.);
#4518=B_SPLINE_CURVE_WITH_KNOTS('',3,(#186923,#186924,#186925,#186926,#186927,
#186928,#186929,#186930,#186931,#186932,#186933,#186934,#186935,#186936,
#186937,#186938,#186939,#186940,#186941,#186942,#186943,#186944,#186945,
#186946,#186947,#186948,#186949,#186950,#186951,#186952,#186953,#186954,
#186955,#186956,#186957,#186958,#186959,#186960,#186961,#186962,#186963,
#186964,#186965,#186966,#186967,#186968,#186969,#186970,#186971,#186972,
#186973,#186974),.UNSPECIFIED.,.F.,.F.,(4,3,3,3,3,3,3,3,3,3,3,3,3,3,3,3,
3,4),(0.,4.29652152201144E-5,8.44519107599058E-5,0.000123669830872989,0.000159788877367001,
0.000170558847912645,0.000181218775907183,0.000181960046452432,0.000214460062643515,
0.000244755726198189,0.000255838271868953,0.000258503253867588,0.000261084955178765,
0.000289370476647358,0.000301101325502013,0.000321109510663637,0.000331113603244449,
0.000341117695825262),.UNSPECIFIED.);
#4519=B_SPLINE_CURVE_WITH_KNOTS('',3,(#186976,#186977,#186978,#186979,#186980,
#186981,#186982,#186983,#186984,#186985,#186986,#186987,#186988,#186989,
#186990,#186991,#186992,#186993,#186994,#186995,#186996,#186997,#186998,
#186999,#187000,#187001,#187002,#187003,#187004,#187005,#187006,#187007,
#187008,#187009,#187010,#187011,#187012,#187013,#187014,#187015,#187016,
#187017,#187018,#187019,#187020,#187021,#187022,#187023,#187024,#187025,
#187026,#187027),.UNSPECIFIED.,.F.,.F.,(4,3,3,3,3,3,3,3,3,3,3,3,3,3,3,3,
3,4),(1.20185167898973E-17,4.30706237879685E-5,8.4741708771448E-5,0.000124159989208214,
0.000160467076293205,0.000170998382116688,0.000182414994733758,0.000213747977645861,
0.000242415955904577,0.000256497573175034,0.000259169422895607,0.000261757777312412,
0.000289965130402962,0.000301877270772896,0.000321937017503138,0.000326951954185698,
0.000334474359209539,0.00034199676423338),.UNSPECIFIED.);
#4520=B_SPLINE_CURVE_WITH_KNOTS('',3,(#187028,#187029,#187030,#187031,#187032,
#187033,#187034,#187035,#187036,#187037,#187038,#187039,#187040,#187041,
#187042,#187043,#187044,#187045,#187046,#187047,#187048,#187049,#187050,
#187051,#187052,#187053,#187054,#187055,#187056,#187057,#187058,#187059,
#187060,#187061,#187062,#187063,#187064,#187065,#187066,#187067,#187068,
#187069,#187070,#187071,#187072,#187073,#187074,#187075,#187076,#187077,
#187078,#187079),.UNSPECIFIED.,.F.,.F.,(4,3,3,3,3,3,3,3,3,3,3,3,3,3,3,3,
3,4),(0.,2.58457451685695E-5,4.25394446195858E-5,6.46659869687149E-5,7.57292581432795E-5,
8.12608937305618E-5,8.26438026273824E-5,8.67925293178441E-5,0.000116015624427412,
0.000130188793976766,0.000151886926306227,0.000161963651211282,0.000162735992470958,
0.000173585058635688,0.000212487880459148,0.000255238173507998,0.000301397761141145,
0.000347170117271364),.UNSPECIFIED.);
#4521=B_SPLINE_CURVE_WITH_KNOTS('',3,(#187081,#187082,#187083,#187084,#187085,
#187086,#187087,#187088,#187089,#187090,#187091,#187092,#187093,#187094,
#187095,#187096,#187097,#187098,#187099,#187100,#187101,#187102,#187103,
#187104,#187105,#187106,#187107,#187108,#187109,#187110,#187111,#187112,
#187113,#187114,#187115,#187116,#187117,#187118,#187119,#187120,#187121,
#187122,#187123,#187124,#187125,#187126),.UNSPECIFIED.,.F.,.F.,(4,3,3,3,
3,3,3,3,3,3,3,3,3,3,3,4),(0.,2.57218162002906E-5,4.2156832256782E-5,6.4587331461703E-5,
7.58025810641635E-5,8.14102058653938E-5,8.28121120657014E-5,8.70178306666241E-5,
0.0001160819556579,0.000130526745999936,0.000162394111022055,0.000174035661333248,
0.000213138396956627,0.00025611693543044,0.000302406662850497,0.000348071322666479),
 .UNSPECIFIED.);
#4522=B_SPLINE_CURVE_WITH_KNOTS('',3,(#187127,#187128,#187129,#187130,#187131,
#187132,#187133,#187134,#187135,#187136,#187137,#187138,#187139,#187140,
#187141,#187142,#187143,#187144,#187145,#187146,#187147,#187148,#187149,
#187150,#187151,#187152,#187153,#187154,#187155,#187156,#187157,#187158,
#187159,#187160,#187161,#187162,#187163,#187164,#187165,#187166,#187167,
#187168,#187169,#187170,#187171,#187172,#187173,#187174,#187175,#187176,
#187177,#187178),.UNSPECIFIED.,.F.,.F.,(4,3,3,3,3,3,3,3,3,3,3,3,3,3,3,3,
3,4),(0.,4.29652152158326E-5,8.4451910753004E-5,0.000123669830864426,0.0001597888773574,
0.000170558847912627,0.000181218775907167,0.000181960046452397,0.000214460062643843,
0.000244755726198955,0.000255838271868947,0.000258503253867582,0.00026108495517876,
0.000289370476648254,0.000301101325502013,0.00032110951066364,0.000331113603244453,
0.000341117695825267),.UNSPECIFIED.);
#4523=B_SPLINE_CURVE_WITH_KNOTS('',3,(#187180,#187181,#187182,#187183,#187184,
#187185,#187186,#187187,#187188,#187189,#187190,#187191,#187192,#187193,
#187194,#187195,#187196,#187197,#187198,#187199,#187200,#187201,#187202,
#187203,#187204,#187205,#187206,#187207,#187208,#187209,#187210,#187211,
#187212,#187213,#187214,#187215,#187216,#187217,#187218,#187219,#187220,
#187221,#187222,#187223,#187224,#187225,#187226,#187227,#187228,#187229,
#187230,#187231),.UNSPECIFIED.,.F.,.F.,(4,3,3,3,3,3,3,3,3,3,3,3,3,3,3,3,
3,4),(0.,4.30706237868942E-5,8.474170876963E-5,0.000124159989205747,0.000160467076290168,
0.000170998382116697,0.000182414994733784,0.000213747977645871,0.000242415955904234,
0.000256497573175044,0.000259169422895617,0.000261757777312423,0.000289965130401751,
0.000301877270772907,0.000321937017503149,0.000326951954185709,0.00033447435920955,
0.000341996764233391),.UNSPECIFIED.);
#4524=B_SPLINE_CURVE_WITH_KNOTS('',3,(#187232,#187233,#187234,#187235,#187236,
#187237,#187238,#187239,#187240,#187241,#187242,#187243,#187244,#187245,
#187246,#187247,#187248,#187249,#187250,#187251,#187252,#187253,#187254,
#187255,#187256,#187257,#187258,#187259,#187260,#187261,#187262,#187263,
#187264,#187265,#187266,#187267,#187268,#187269,#187270,#187271,#187272,
#187273,#187274,#187275,#187276,#187277,#187278,#187279,#187280,#187281,
#187282,#187283),.UNSPECIFIED.,.F.,.F.,(4,3,3,3,3,3,3,3,3,3,3,3,3,3,3,3,
3,4),(0.,2.58457451695845E-5,4.25394446195289E-5,6.46659869686875E-5,7.57292581432667E-5,
8.12608937305564E-5,8.26438026273788E-5,8.6792529317846E-5,0.000116015624427563,
0.000130188793976769,0.000151886926306231,0.000161963651211295,0.000162735992470961,
0.000173585058635692,0.000212487880462759,0.00025523817351527,0.000301397761152659,
0.000347170117271367),.UNSPECIFIED.);
#4525=B_SPLINE_CURVE_WITH_KNOTS('',3,(#187285,#187286,#187287,#187288,#187289,
#187290,#187291,#187292,#187293,#187294,#187295,#187296,#187297,#187298,
#187299,#187300,#187301,#187302,#187303,#187304,#187305,#187306,#187307,
#187308,#187309,#187310,#187311,#187312,#187313,#187314,#187315,#187316,
#187317,#187318,#187319,#187320,#187321,#187322,#187323,#187324,#187325,
#187326,#187327,#187328,#187329,#187330),.UNSPECIFIED.,.F.,.F.,(4,3,3,3,
3,3,3,3,3,3,3,3,3,3,3,4),(0.,2.57218161974927E-5,4.21568322567519E-5,6.45873314616843E-5,
7.58025810641505E-5,8.14102058653837E-5,8.28121120656919E-5,8.70178306666168E-5,
0.000116081955657236,0.000130526745999925,0.000162394111022051,0.000174035661333234,
0.000213138396959219,0.000256116935435569,0.000302406662858305,0.000348071322666466),
 .UNSPECIFIED.);
#4526=B_SPLINE_CURVE_WITH_KNOTS('',3,(#187331,#187332,#187333,#187334,#187335,
#187336,#187337,#187338,#187339,#187340,#187341,#187342,#187343,#187344,
#187345,#187346,#187347,#187348,#187349,#187350,#187351,#187352,#187353,
#187354,#187355,#187356,#187357,#187358,#187359,#187360,#187361,#187362,
#187363,#187364,#187365,#187366,#187367,#187368,#187369,#187370,#187371,
#187372,#187373,#187374,#187375,#187376,#187377,#187378,#187379,#187380,
#187381,#187382),.UNSPECIFIED.,.F.,.F.,(4,3,3,3,3,3,3,3,3,3,3,3,3,3,3,3,
3,4),(0.,4.29652152193347E-5,8.4451910758867E-5,0.000123669830872074,0.000159788877366483,
0.000170558847912628,0.000181218775907168,0.000181960046452402,0.000214460062643761,
0.00024475572619894,0.000255838271868948,0.000258503253867583,0.000261084955178761,
0.00028937047664693,0.000301101325502014,0.000321109510663641,0.000331113603244454,
0.000341117695825268),.UNSPECIFIED.);
#4527=B_SPLINE_CURVE_WITH_KNOTS('',3,(#187384,#187385,#187386,#187387,#187388,
#187389,#187390,#187391,#187392,#187393,#187394,#187395,#187396,#187397,
#187398,#187399,#187400,#187401,#187402,#187403,#187404,#187405,#187406,
#187407,#187408,#187409,#187410,#187411,#187412,#187413,#187414,#187415,
#187416,#187417,#187418,#187419,#187420,#187421,#187422,#187423,#187424,
#187425,#187426,#187427,#187428,#187429,#187430,#187431,#187432,#187433,
#187434,#187435),.UNSPECIFIED.,.F.,.F.,(4,3,3,3,3,3,3,3,3,3,3,3,3,3,3,3,
3,4),(0.,4.30706237884788E-5,8.47417087722986E-5,0.000124159989209235,0.000160467076294441,
0.000170998382116698,0.00018241499473378,0.000213747977645868,0.000242415955903622,
0.000256497573175039,0.000259169422895612,0.000261757777312418,0.000289965130403898,
0.000301877270772899,0.00032193701750314,0.0003269519541857,0.00033447435920954,
0.00034199676423338),.UNSPECIFIED.);
#4528=B_SPLINE_CURVE_WITH_KNOTS('',3,(#187436,#187437,#187438,#187439,#187440,
#187441,#187442,#187443,#187444,#187445,#187446,#187447,#187448,#187449,
#187450,#187451,#187452,#187453,#187454,#187455,#187456,#187457,#187458,
#187459,#187460,#187461,#187462,#187463,#187464,#187465,#187466,#187467,
#187468,#187469,#187470,#187471,#187472,#187473,#187474,#187475,#187476,
#187477,#187478,#187479,#187480,#187481,#187482,#187483,#187484,#187485,
#187486,#187487),.UNSPECIFIED.,.F.,.F.,(4,3,3,3,3,3,3,3,3,3,3,3,3,3,3,3,
3,4),(0.,2.58457451704755E-5,4.25394446194672E-5,6.46659869686538E-5,7.57292581432472E-5,
8.12608937305438E-5,8.2643802627368E-5,8.67925293178405E-5,0.000116015624427198,
0.000130188793976761,0.000151886926306221,0.000161963651211268,0.000162735992470951,
0.000173585058635681,0.000212487880458066,0.000255238173506561,0.000301397761140657,
0.000347170117271375),.UNSPECIFIED.);
#4529=B_SPLINE_CURVE_WITH_KNOTS('',3,(#187489,#187490,#187491,#187492,#187493,
#187494,#187495,#187496,#187497,#187498,#187499,#187500,#187501,#187502,
#187503,#187504,#187505,#187506,#187507,#187508,#187509,#187510,#187511,
#187512,#187513,#187514,#187515,#187516,#187517,#187518,#187519,#187520,
#187521,#187522,#187523,#187524,#187525,#187526,#187527,#187528,#187529,
#187530,#187531,#187532,#187533,#187534),.UNSPECIFIED.,.F.,.F.,(4,3,3,3,
3,3,3,3,3,3,3,3,3,3,3,4),(0.,2.57218162000528E-5,4.2156832256754E-5,6.45873314616856E-5,
7.58025810641514E-5,8.14102058653844E-5,8.28121120656926E-5,8.70178306666173E-5,
0.00011608195565755,0.000130526745999926,0.000162394111022041,0.000174035661333235,
0.000213138396956922,0.000256116935431229,0.000302406662852368,0.000348071322666458),
 .UNSPECIFIED.);
#4530=B_SPLINE_CURVE_WITH_KNOTS('',3,(#187535,#187536,#187537,#187538,#187539,
#187540,#187541,#187542,#187543,#187544,#187545,#187546,#187547,#187548,
#187549,#187550,#187551,#187552,#187553,#187554,#187555,#187556,#187557,
#187558,#187559,#187560,#187561,#187562,#187563,#187564,#187565,#187566,
#187567,#187568,#187569,#187570,#187571,#187572,#187573,#187574,#187575,
#187576,#187577,#187578,#187579,#187580,#187581,#187582,#187583,#187584,
#187585,#187586),.UNSPECIFIED.,.F.,.F.,(4,3,3,3,3,3,3,3,3,3,3,3,3,3,3,3,
3,4),(0.,4.29652152177208E-5,8.44519107561497E-5,0.000123669830868545,0.000159788877362415,
0.00017055884791262,0.00018121877590716,0.000181960046452397,0.000214460062643471,
0.000244755726198109,0.000255838271868942,0.000258503253867577,0.000261084955178755,
0.000289370476648085,0.00030110132550201,0.000321109510663637,0.000331113603244451,
0.000341117695825265),.UNSPECIFIED.);
#4531=B_SPLINE_CURVE_WITH_KNOTS('',3,(#187588,#187589,#187590,#187591,#187592,
#187593,#187594,#187595,#187596,#187597,#187598,#187599,#187600,#187601,
#187602,#187603,#187604,#187605,#187606,#187607,#187608,#187609,#187610,
#187611,#187612,#187613,#187614,#187615,#187616,#187617,#187618,#187619,
#187620,#187621,#187622,#187623,#187624,#187625,#187626,#187627,#187628,
#187629,#187630,#187631,#187632,#187633,#187634,#187635,#187636,#187637,
#187638,#187639),.UNSPECIFIED.,.F.,.F.,(4,3,3,3,3,3,3,3,3,3,3,3,3,3,3,3,
3,4),(0.,4.30706237855123E-5,8.47417087672605E-5,0.000124159989202624,0.000160467076286203,
0.000170998382116679,0.000182414994733753,0.000213747977645857,0.000242415955904274,
0.000256497573175035,0.000259169422895609,0.000261757777312415,0.000289965130404309,
0.000301877270772903,0.000321937017503147,0.000326951954185708,0.00033447435920955,
0.000341996764233392),.UNSPECIFIED.);
#4532=B_SPLINE_CURVE_WITH_KNOTS('',3,(#187640,#187641,#187642,#187643,#187644,
#187645,#187646,#187647,#187648,#187649,#187650,#187651,#187652,#187653,
#187654,#187655,#187656,#187657,#187658,#187659,#187660,#187661,#187662,
#187663,#187664,#187665,#187666,#187667,#187668,#187669,#187670,#187671,
#187672,#187673,#187674,#187675,#187676,#187677,#187678,#187679,#187680,
#187681,#187682,#187683,#187684,#187685,#187686,#187687,#187688,#187689,
#187690,#187691),.UNSPECIFIED.,.F.,.F.,(4,3,3,3,3,3,3,3,3,3,3,3,3,3,3,3,
3,4),(6.93889390390723E-18,2.58457451683063E-5,4.25394446195843E-5,6.46659869687167E-5,
7.57292581432828E-5,8.12608937305659E-5,8.26438026273867E-5,8.6792529317849E-5,
0.000116015624427382,0.00013018879397677,0.000151886926306231,0.000161963651211302,
0.000162735992470961,0.000173585058635691,0.000212487880461466,0.000255238173511805,
0.000301397761145146,0.000347170117271358),.UNSPECIFIED.);
#4533=B_SPLINE_CURVE_WITH_KNOTS('',3,(#187693,#187694,#187695,#187696,#187697,
#187698,#187699,#187700,#187701,#187702,#187703,#187704,#187705,#187706,
#187707,#187708,#187709,#187710,#187711,#187712,#187713,#187714,#187715,
#187716,#187717,#187718,#187719,#187720,#187721,#187722,#187723,#187724,
#187725,#187726,#187727,#187728,#187729,#187730,#187731,#187732,#187733,
#187734,#187735,#187736,#187737,#187738),.UNSPECIFIED.,.F.,.F.,(4,3,3,3,
3,3,3,3,3,3,3,3,3,3,3,4),(6.93889390390723E-18,2.57218161972534E-5,4.2156832256757E-5,
6.458733146169E-5,7.58025810641566E-5,8.14102058653898E-5,8.28121120656981E-5,
8.70178306666231E-5,0.000116081955657329,0.000130526745999931,0.000162394111022074,
0.000174035661333239,0.000213138396957694,0.000256116935432815,0.000302406662854965,
0.000348071322666459),.UNSPECIFIED.);
#4534=B_SPLINE_CURVE_WITH_KNOTS('',3,(#187739,#187740,#187741,#187742,#187743,
#187744,#187745,#187746,#187747,#187748,#187749,#187750,#187751,#187752,
#187753,#187754,#187755,#187756,#187757,#187758,#187759,#187760,#187761,
#187762,#187763,#187764,#187765,#187766,#187767,#187768,#187769,#187770,
#187771,#187772,#187773,#187774,#187775,#187776,#187777,#187778,#187779,
#187780,#187781,#187782,#187783,#187784,#187785,#187786,#187787,#187788,
#187789,#187790),.UNSPECIFIED.,.F.,.F.,(4,3,3,3,3,3,3,3,3,3,3,3,3,3,3,3,
3,4),(0.,4.2965215221334E-5,8.44519107622145E-5,0.000123669830876504,0.000159788877371945,
0.000170558847912634,0.000181218775907173,0.000181960046452426,0.000214460062644004,
0.0002447557261995,0.000255838271868948,0.000258503253867583,0.000261084955178761,
0.000289370476645958,0.000301101325502012,0.000321109510663638,0.000331113603244451,
0.000341117695825263),.UNSPECIFIED.);
#4535=B_SPLINE_CURVE_WITH_KNOTS('',3,(#187792,#187793,#187794,#187795,#187796,
#187797,#187798,#187799,#187800,#187801,#187802,#187803,#187804,#187805,
#187806,#187807,#187808,#187809,#187810,#187811,#187812,#187813,#187814,
#187815,#187816,#187817,#187818,#187819,#187820,#187821,#187822,#187823,
#187824,#187825,#187826,#187827,#187828,#187829,#187830,#187831,#187832,
#187833,#187834,#187835,#187836,#187837,#187838,#187839,#187840,#187841,
#187842,#187843),.UNSPECIFIED.,.F.,.F.,(4,3,3,3,3,3,3,3,3,3,3,3,3,3,3,3,
3,4),(0.,4.30706237842057E-5,8.47417087648121E-5,0.000124159989199012,0.000160467076281244,
0.000170998382116703,0.000182414994733766,0.000213747977645878,0.00024241595590268,
0.000256497573175052,0.000259169422895626,0.000261757777312431,0.000289965130404317,
0.000301877270772916,0.000321937017503159,0.00032695195418572,0.000334474359209561,
0.000341996764233402),.UNSPECIFIED.);
#4536=B_SPLINE_CURVE_WITH_KNOTS('',3,(#187844,#187845,#187846,#187847,#187848,
#187849,#187850,#187851,#187852,#187853,#187854,#187855,#187856,#187857,
#187858,#187859,#187860,#187861,#187862,#187863,#187864,#187865,#187866,
#187867,#187868,#187869,#187870,#187871,#187872,#187873,#187874,#187875,
#187876,#187877,#187878,#187879,#187880,#187881,#187882,#187883,#187884,
#187885,#187886,#187887,#187888,#187889,#187890,#187891,#187892,#187893,
#187894,#187895),.UNSPECIFIED.,.F.,.F.,(4,3,3,3,3,3,3,3,3,3,3,3,3,3,3,3,
3,4),(3.46944695195361E-18,2.58457451697369E-5,4.25394446196474E-5,6.46659869687486E-5,
7.57292581432992E-5,8.12608937305745E-5,8.26438026273933E-5,8.67925293178498E-5,
0.0001160156244268,0.000130188793976773,0.000151886926306235,0.000161963651211278,
0.000162735992470965,0.000173585058635696,0.000212487880457896,0.000255238173505114,
0.000301397761135914,0.000347170117271375),.UNSPECIFIED.);
#4537=B_SPLINE_CURVE_WITH_KNOTS('',3,(#187897,#187898,#187899,#187900,#187901,
#187902,#187903,#187904,#187905,#187906,#187907,#187908,#187909,#187910,
#187911,#187912,#187913,#187914,#187915,#187916,#187917,#187918,#187919,
#187920,#187921,#187922,#187923,#187924,#187925,#187926,#187927,#187928,
#187929,#187930,#187931,#187932,#187933,#187934,#187935,#187936,#187937,
#187938,#187939,#187940,#187941,#187942),.UNSPECIFIED.,.F.,.F.,(4,3,3,3,
3,3,3,3,3,3,3,3,3,3,3,4),(0.,2.57218161993105E-5,4.21568322568682E-5,6.45873314617395E-5,
7.58025810641752E-5,8.1410205865393E-5,8.28121120656975E-5,8.70178306666108E-5,
0.000116081955657196,0.000130526745999916,0.000162394111022044,0.000174035661333222,
0.000213138396958914,0.000256116935435134,0.000302406662858135,0.000348071322666431),
 .UNSPECIFIED.);
#4538=B_SPLINE_CURVE_WITH_KNOTS('',3,(#187943,#187944,#187945,#187946,#187947,
#187948,#187949,#187950,#187951,#187952,#187953,#187954,#187955,#187956,
#187957,#187958,#187959,#187960,#187961,#187962,#187963,#187964,#187965,
#187966,#187967,#187968,#187969,#187970,#187971,#187972,#187973,#187974,
#187975,#187976,#187977,#187978,#187979,#187980,#187981,#187982,#187983,
#187984,#187985,#187986,#187987,#187988,#187989,#187990,#187991,#187992,
#187993,#187994),.UNSPECIFIED.,.F.,.F.,(4,3,3,3,3,3,3,3,3,3,3,3,3,3,3,3,
3,4),(0.,4.29652152131072E-5,8.44519107485544E-5,0.000123669830858988,0.000159788877351408,
0.000170558847912628,0.000181218775907167,0.00018196004645239,0.000214460062642862,
0.000244755726196479,0.00025583827186894,0.000258503253867575,0.000261084955178753,
0.000289370476649787,0.000301101325502002,0.000321109510663627,0.00033111360324444,
0.000341117695825252),.UNSPECIFIED.);
#4539=B_SPLINE_CURVE_WITH_KNOTS('',3,(#187996,#187997,#187998,#187999,#188000,
#188001,#188002,#188003,#188004,#188005,#188006,#188007,#188008,#188009,
#188010,#188011,#188012,#188013,#188014,#188015,#188016,#188017,#188018,
#188019,#188020,#188021,#188022,#188023,#188024,#188025,#188026,#188027,
#188028,#188029,#188030,#188031,#188032,#188033,#188034,#188035,#188036,
#188037,#188038,#188039,#188040,#188041,#188042,#188043,#188044,#188045,
#188046,#188047),.UNSPECIFIED.,.F.,.F.,(4,3,3,3,3,3,3,3,3,3,3,3,3,3,3,3,
3,4),(0.,4.30706237861054E-5,8.47417087681986E-5,0.000124159989203905,0.000160467076287747,
0.000170998382116685,0.000182414994733779,0.000213747977645861,0.000242415955902392,
0.000256497573175037,0.000259169422895611,0.000261757777312416,0.000289965130404567,
0.000301877270772903,0.000321937017503146,0.000326951954185707,0.000334474359209548,
0.000341996764233389),.UNSPECIFIED.);
#4540=B_SPLINE_CURVE_WITH_KNOTS('',3,(#188048,#188049,#188050,#188051,#188052,
#188053,#188054,#188055,#188056,#188057,#188058,#188059,#188060,#188061,
#188062,#188063,#188064,#188065,#188066,#188067,#188068,#188069,#188070,
#188071,#188072,#188073,#188074,#188075,#188076,#188077,#188078,#188079,
#188080,#188081,#188082,#188083,#188084,#188085,#188086,#188087,#188088,
#188089,#188090,#188091,#188092,#188093,#188094,#188095,#188096,#188097,
#188098,#188099),.UNSPECIFIED.,.F.,.F.,(4,3,3,3,3,3,3,3,3,3,3,3,3,3,3,3,
3,4),(3.46944695195361E-18,2.58457451678929E-5,4.25394446195445E-5,6.46659869686953E-5,
7.57292581432707E-5,8.12608937305584E-5,8.26438026273803E-5,8.67925293178461E-5,
0.000116015624426703,0.000130188793976767,0.000151886926306228,0.000161963651211296,
0.000162735992470958,0.000173585058635689,0.00021248788045957,0.000255238173508425,
0.000301397761140786,0.000347170117271359),.UNSPECIFIED.);
#4541=B_SPLINE_CURVE_WITH_KNOTS('',3,(#188101,#188102,#188103,#188104,#188105,
#188106,#188107,#188108,#188109,#188110,#188111,#188112,#188113,#188114,
#188115,#188116,#188117,#188118,#188119,#188120,#188121,#188122,#188123,
#188124,#188125,#188126,#188127,#188128,#188129,#188130,#188131,#188132,
#188133,#188134,#188135,#188136,#188137,#188138,#188139,#188140,#188141,
#188142,#188143,#188144,#188145,#188146),.UNSPECIFIED.,.F.,.F.,(4,3,3,3,
3,3,3,3,3,3,3,3,3,3,3,4),(0.,2.57218162010215E-5,4.21568322568023E-5,6.45873314617128E-5,
7.5802581064168E-5,8.14102058653956E-5,8.28121120657025E-5,8.70178306666232E-5,
0.000116081955658569,0.000130526745999935,0.000162394111022054,0.000174035661333246,
0.000213138396958572,0.000256116935434451,0.000302406662857123,0.000348071322666499),
 .UNSPECIFIED.);
#4542=B_SPLINE_CURVE_WITH_KNOTS('',3,(#188147,#188148,#188149,#188150,#188151,
#188152,#188153,#188154,#188155,#188156,#188157,#188158,#188159,#188160,
#188161,#188162,#188163,#188164,#188165,#188166,#188167,#188168,#188169,
#188170,#188171,#188172,#188173,#188174,#188175,#188176,#188177,#188178,
#188179,#188180,#188181,#188182,#188183,#188184,#188185,#188186,#188187,
#188188,#188189,#188190,#188191,#188192,#188193,#188194,#188195,#188196,
#188197,#188198),.UNSPECIFIED.,.F.,.F.,(4,3,3,3,3,3,3,3,3,3,3,3,3,3,3,3,
3,4),(0.,4.2965215210667E-5,8.44519107445277E-5,0.000123669830853843,0.000159788877345156,
0.000170558847912632,0.000181218775907172,0.000181960046452383,0.000214460062643245,
0.000244755726197489,0.000255838271868954,0.000258503253867589,0.000261084955178766,
0.000289370476648082,0.000301101325502021,0.000321109510663648,0.000331113603244462,
0.000341117695825276),.UNSPECIFIED.);
#4543=B_SPLINE_CURVE_WITH_KNOTS('',3,(#188200,#188201,#188202,#188203,#188204,
#188205,#188206,#188207,#188208,#188209,#188210,#188211,#188212,#188213,
#188214,#188215,#188216,#188217,#188218,#188219,#188220,#188221,#188222,
#188223,#188224,#188225,#188226,#188227,#188228,#188229,#188230,#188231,
#188232,#188233,#188234,#188235,#188236,#188237,#188238,#188239,#188240,
#188241,#188242,#188243,#188244,#188245,#188246,#188247,#188248,#188249,
#188250,#188251),.UNSPECIFIED.,.F.,.F.,(4,3,3,3,3,3,3,3,3,3,3,3,3,3,3,3,
3,4),(0.,4.30706237856851E-5,8.47417087672796E-5,0.000124159989202264,0.000160467076285325,
0.000170998382116702,0.000182414994733779,0.000213747977645874,0.000242415955903721,
0.000256497573175046,0.00025916942289562,0.000261757777312425,0.000289965130403,
0.000301877270772908,0.000321937017503149,0.00032695195418571,0.00033447435920955,
0.000341996764233391),.UNSPECIFIED.);
#4544=B_SPLINE_CURVE_WITH_KNOTS('',3,(#188252,#188253,#188254,#188255,#188256,
#188257,#188258,#188259,#188260,#188261,#188262,#188263,#188264,#188265,
#188266,#188267,#188268,#188269,#188270,#188271,#188272,#188273,#188274,
#188275,#188276,#188277,#188278,#188279,#188280,#188281,#188282,#188283,
#188284,#188285,#188286,#188287,#188288,#188289,#188290,#188291,#188292,
#188293,#188294,#188295,#188296,#188297,#188298,#188299,#188300,#188301,
#188302,#188303),.UNSPECIFIED.,.F.,.F.,(4,3,3,3,3,3,3,3,3,3,3,3,3,3,3,3,
3,4),(3.46944695195361E-18,2.58457451677859E-5,4.2539444619544E-5,6.46659869686969E-5,
7.57292581432733E-5,8.12608937305615E-5,8.26438026273836E-5,8.67925293178497E-5,
0.000116015624427814,0.000130188793976773,0.000151886926306234,0.000161963651211293,
0.000162735992470965,0.000173585058635696,0.00021248788046203,0.000255238173515158,
0.000301397761155678,0.000347170117271372),.UNSPECIFIED.);
#4545=B_SPLINE_CURVE_WITH_KNOTS('',3,(#188305,#188306,#188307,#188308,#188309,
#188310,#188311,#188312,#188313,#188314,#188315,#188316,#188317,#188318,
#188319,#188320,#188321,#188322,#188323,#188324,#188325,#188326,#188327,
#188328,#188329,#188330,#188331,#188332,#188333,#188334,#188335,#188336,
#188337,#188338,#188339,#188340,#188341,#188342,#188343,#188344,#188345,
#188346,#188347,#188348,#188349,#188350),.UNSPECIFIED.,.F.,.F.,(4,3,3,3,
3,3,3,3,3,3,3,3,3,3,3,4),(0.,2.57218161992883E-5,4.21568322568875E-5,6.45873314617512E-5,
7.5802581064183E-5,8.14102058653989E-5,8.28121120657029E-5,8.70178306666148E-5,
0.000116081955658576,0.000130526745999922,0.00016239411102203,0.00017403566133323,
0.000213138396955947,0.000256116935429326,0.000302406662849522,0.000348071322666453),
 .UNSPECIFIED.);
#4546=B_SPLINE_CURVE_WITH_KNOTS('',3,(#188351,#188352,#188353,#188354,#188355,
#188356,#188357,#188358,#188359,#188360,#188361,#188362,#188363,#188364,
#188365,#188366,#188367,#188368,#188369,#188370,#188371,#188372,#188373,
#188374,#188375,#188376,#188377,#188378,#188379,#188380,#188381,#188382,
#188383,#188384,#188385,#188386,#188387,#188388,#188389,#188390,#188391,
#188392,#188393,#188394,#188395,#188396,#188397,#188398,#188399,#188400,
#188401,#188402),.UNSPECIFIED.,.F.,.F.,(4,3,3,3,3,3,3,3,3,3,3,3,3,3,3,3,
3,4),(0.,4.29652152159528E-5,8.44519107530115E-5,0.000123669830864204,0.000159788877356665,
0.000170558847912628,0.000181218775907167,0.000181960046452395,0.000214460062643637,
0.000244755726198709,0.00025583827186894,0.000258503253867575,0.000261084955178752,
0.000289370476647891,0.000301101325502002,0.000321109510663627,0.00033111360324444,
0.000341117695825252),.UNSPECIFIED.);
#4547=B_SPLINE_CURVE_WITH_KNOTS('',3,(#188404,#188405,#188406,#188407,#188408,
#188409,#188410,#188411,#188412,#188413,#188414,#188415,#188416,#188417,
#188418,#188419,#188420,#188421,#188422,#188423,#188424,#188425,#188426,
#188427,#188428,#188429,#188430,#188431,#188432,#188433,#188434,#188435,
#188436,#188437,#188438,#188439,#188440,#188441,#188442,#188443,#188444,
#188445,#188446,#188447,#188448,#188449,#188450,#188451,#188452,#188453,
#188454,#188455),.UNSPECIFIED.,.F.,.F.,(4,3,3,3,3,3,3,3,3,3,3,3,3,3,3,3,
3,4),(0.,4.3070623787178E-5,8.47417087700662E-5,0.000124159989206384,0.000160467076290823,
0.000170998382116695,0.000182414994733763,0.000213747977645866,0.000242415955903335,
0.000256497573175037,0.00025916942289561,0.000261757777312416,0.000289965130403811,
0.000301877270772898,0.000321937017503139,0.000326951954185699,0.00033447435920954,
0.00034199676423338),.UNSPECIFIED.);
#4548=B_SPLINE_CURVE_WITH_KNOTS('',3,(#188456,#188457,#188458,#188459,#188460,
#188461,#188462,#188463,#188464,#188465,#188466,#188467,#188468,#188469,
#188470,#188471,#188472,#188473,#188474,#188475,#188476,#188477,#188478,
#188479,#188480,#188481,#188482,#188483,#188484,#188485,#188486,#188487,
#188488,#188489,#188490,#188491,#188492,#188493,#188494,#188495,#188496,
#188497,#188498,#188499,#188500,#188501,#188502,#188503,#188504,#188505,
#188506,#188507),.UNSPECIFIED.,.F.,.F.,(4,3,3,3,3,3,3,3,3,3,3,3,3,3,3,3,
3,4),(0.,2.58457451688714E-5,4.25394446196352E-5,6.46659869687418E-5,7.5729258143295E-5,
8.12608937305717E-5,8.26438026273908E-5,8.67925293178483E-5,0.000116015624427734,
0.000130188793976772,0.000151886926306235,0.000161963651211294,0.000162735992470966,
0.000173585058635697,0.000212487880462616,0.000255238173515711,0.000301397761155049,
0.000347170117271365),.UNSPECIFIED.);
#4549=B_SPLINE_CURVE_WITH_KNOTS('',3,(#188509,#188510,#188511,#188512,#188513,
#188514,#188515,#188516,#188517,#188518,#188519,#188520,#188521,#188522,
#188523,#188524,#188525,#188526,#188527,#188528,#188529,#188530,#188531,
#188532,#188533,#188534,#188535,#188536,#188537,#188538,#188539,#188540,
#188541,#188542,#188543,#188544,#188545,#188546,#188547,#188548,#188549,
#188550,#188551,#188552,#188553,#188554),.UNSPECIFIED.,.F.,.F.,(4,3,3,3,
3,3,3,3,3,3,3,3,3,3,3,4),(0.,2.57218162002632E-5,4.21568322568512E-5,6.45873314617311E-5,
7.58025810641711E-5,8.1410205865391E-5,8.2812112065696E-5,8.7017830666611E-5,
0.000116081955658825,0.000130526745999917,0.000162394111022047,0.000174035661333222,
0.000213138396959396,0.000256116935436168,0.000302406662860064,0.000348071322666447),
 .UNSPECIFIED.);
#4550=B_SPLINE_CURVE_WITH_KNOTS('',3,(#188555,#188556,#188557,#188558,#188559,
#188560,#188561,#188562,#188563,#188564,#188565,#188566,#188567,#188568,
#188569,#188570,#188571,#188572,#188573,#188574,#188575,#188576,#188577,
#188578,#188579,#188580,#188581,#188582,#188583,#188584,#188585,#188586,
#188587,#188588,#188589,#188590,#188591,#188592,#188593,#188594,#188595,
#188596,#188597,#188598,#188599,#188600,#188601,#188602,#188603,#188604,
#188605,#188606),.UNSPECIFIED.,.F.,.F.,(4,3,3,3,3,3,3,3,3,3,3,3,3,3,3,3,
3,4),(0.,4.29652152163955E-5,8.44519107540137E-5,0.000123669830865945,0.000159788877359403,
0.000170558847912639,0.000181218775907178,0.00018196004645242,0.00021446006264403,
0.000244755726199579,0.000255838271868947,0.000258503253867582,0.000261084955178759,
0.0002893704766472,0.000301101325502007,0.000321109510663631,0.000331113603244444,
0.000341117695825256),.UNSPECIFIED.);
#4551=B_SPLINE_CURVE_WITH_KNOTS('',3,(#188608,#188609,#188610,#188611,#188612,
#188613,#188614,#188615,#188616,#188617,#188618,#188619,#188620,#188621,
#188622,#188623,#188624,#188625,#188626,#188627,#188628,#188629,#188630,
#188631,#188632,#188633,#188634,#188635,#188636,#188637,#188638,#188639,
#188640,#188641,#188642,#188643,#188644,#188645,#188646,#188647,#188648,
#188649,#188650,#188651,#188652,#188653,#188654,#188655,#188656,#188657,
#188658,#188659),.UNSPECIFIED.,.F.,.F.,(4,3,3,3,3,3,3,3,3,3,3,3,3,3,3,3,
3,4),(0.,4.30706237872259E-5,8.47417087700833E-5,0.000124159989206224,0.000160467076290431,
0.000170998382116682,0.000182414994733756,0.000213747977645859,0.000242415955905012,
0.000256497573175035,0.000259169422895609,0.000261757777312414,0.000289965130402064,
0.000301877270772901,0.000321937017503145,0.000326951954185706,0.000334474359209547,
0.000341996764233389),.UNSPECIFIED.);
#4552=B_SPLINE_CURVE_WITH_KNOTS('',3,(#188660,#188661,#188662,#188663,#188664,
#188665,#188666,#188667,#188668,#188669,#188670,#188671,#188672,#188673,
#188674,#188675,#188676,#188677,#188678,#188679,#188680,#188681,#188682,
#188683,#188684,#188685,#188686,#188687,#188688,#188689,#188690,#188691,
#188692,#188693,#188694,#188695,#188696,#188697,#188698,#188699,#188700,
#188701,#188702,#188703,#188704,#188705,#188706,#188707,#188708,#188709,
#188710,#188711),.UNSPECIFIED.,.F.,.F.,(4,3,3,3,3,3,3,3,3,3,3,3,3,3,3,3,
3,4),(0.,2.58457451680095E-5,4.2539444619618E-5,6.46659869687305E-5,7.57292581432868E-5,
8.12608937305649E-5,8.26438026273845E-5,8.67925293178431E-5,0.000116015624426959,
0.000130188793976765,0.000151886926306225,0.000161963651211284,0.000162735992470956,
0.000173585058635686,0.000212487880456419,0.000255238173500689,0.000301397761125226,
0.000347170117271373),.UNSPECIFIED.);
#4553=B_SPLINE_CURVE_WITH_KNOTS('',3,(#188713,#188714,#188715,#188716,#188717,
#188718,#188719,#188720,#188721,#188722,#188723,#188724,#188725,#188726,
#188727,#188728,#188729,#188730,#188731,#188732,#188733,#188734,#188735,
#188736,#188737,#188738,#188739,#188740,#188741,#188742,#188743,#188744,
#188745,#188746,#188747,#188748,#188749,#188750,#188751,#188752,#188753,
#188754,#188755,#188756,#188757,#188758),.UNSPECIFIED.,.F.,.F.,(4,3,3,3,
3,3,3,3,3,3,3,3,3,3,3,4),(8.67361737988404E-19,2.57218162009145E-5,4.21568322566762E-5,
6.45873314616513E-5,7.58025810641389E-5,8.14102058653827E-5,8.28121120656936E-5,
8.70178306666264E-5,0.000116081955658878,0.000130526745999939,0.000162394111022056,
0.000174035661333252,0.000213138396958378,0.000256116935433806,0.000302406662855308,
0.000348071322666491),.UNSPECIFIED.);
#4554=B_SPLINE_CURVE_WITH_KNOTS('',3,(#188759,#188760,#188761,#188762,#188763,
#188764,#188765,#188766,#188767,#188768,#188769,#188770,#188771,#188772,
#188773,#188774,#188775,#188776,#188777,#188778,#188779,#188780,#188781,
#188782,#188783,#188784,#188785,#188786,#188787,#188788,#188789,#188790,
#188791,#188792,#188793,#188794,#188795,#188796,#188797,#188798,#188799,
#188800,#188801,#188802,#188803,#188804,#188805,#188806,#188807,#188808,
#188809,#188810),.UNSPECIFIED.,.F.,.F.,(4,3,3,3,3,3,3,3,3,3,3,3,3,3,3,3,
3,4),(0.,4.29652152202514E-5,8.4451910759941E-5,0.000123669830872665,0.000159788877366079,
0.000170558847912629,0.000181218775907169,0.000181960046452395,0.000214460062643499,
0.000244755726198446,0.000255838271868949,0.000258503253867584,0.000261084955178762,
0.000289370476647764,0.000301101325502016,0.000321109510663643,0.000331113603244456,
0.00034111769582527),.UNSPECIFIED.);
#4555=B_SPLINE_CURVE_WITH_KNOTS('',3,(#188812,#188813,#188814,#188815,#188816,
#188817,#188818,#188819,#188820,#188821,#188822,#188823,#188824,#188825,
#188826,#188827,#188828,#188829,#188830,#188831,#188832,#188833,#188834,
#188835,#188836,#188837,#188838,#188839,#188840,#188841,#188842,#188843,
#188844,#188845,#188846,#188847,#188848,#188849,#188850,#188851,#188852,
#188853,#188854,#188855,#188856,#188857,#188858,#188859,#188860,#188861,
#188862,#188863),.UNSPECIFIED.,.F.,.F.,(4,3,3,3,3,3,3,3,3,3,3,3,3,3,3,3,
3,4),(5.96311194867027E-19,4.3070623785328E-5,8.47417087668814E-5,0.000124159989202045,
0.000160467076285363,0.000170998382116684,0.000182414994733754,0.000213747977645859,
0.000242415955902855,0.000256497573175034,0.000259169422895607,0.000261757777312412,
0.000289965130403962,0.000301877270772898,0.00032193701750314,0.000326951954185701,
0.000334474359209542,0.000341996764233383),.UNSPECIFIED.);
#4556=B_SPLINE_CURVE_WITH_KNOTS('',3,(#188864,#188865,#188866,#188867,#188868,
#188869,#188870,#188871,#188872,#188873,#188874,#188875,#188876,#188877,
#188878,#188879,#188880,#188881,#188882,#188883,#188884,#188885,#188886,
#188887,#188888,#188889,#188890,#188891,#188892,#188893,#188894,#188895,
#188896,#188897,#188898,#188899,#188900,#188901,#188902,#188903,#188904,
#188905,#188906,#188907,#188908,#188909,#188910,#188911,#188912,#188913,
#188914,#188915),.UNSPECIFIED.,.F.,.F.,(4,3,3,3,3,3,3,3,3,3,3,3,3,3,3,3,
3,4),(2.76132740804902E-19,2.58457451672193E-5,4.25394446196239E-5,6.46659869687285E-5,
7.57292581432808E-5,8.1260893730557E-5,8.2643802627376E-5,8.67925293178331E-5,
0.000116015624427903,0.00013018879397675,0.000151886926306208,0.000161963651211269,
0.000162735992470937,0.000173585058635666,0.000212487880463427,0.000255238173517339,
0.000301397761157609,0.000347170117271358),.UNSPECIFIED.);
#4557=B_SPLINE_CURVE_WITH_KNOTS('',3,(#188917,#188918,#188919,#188920,#188921,
#188922,#188923,#188924,#188925,#188926,#188927,#188928,#188929,#188930,
#188931,#188932,#188933,#188934,#188935,#188936,#188937,#188938,#188939,
#188940,#188941,#188942,#188943,#188944,#188945,#188946,#188947,#188948,
#188949,#188950,#188951,#188952,#188953,#188954,#188955,#188956,#188957,
#188958,#188959,#188960,#188961,#188962),.UNSPECIFIED.,.F.,.F.,(4,3,3,3,
3,3,3,3,3,3,3,3,3,3,3,4),(2.74438674910393E-19,2.57218161992784E-5,4.21568322568869E-5,
6.45873314617526E-5,7.58025810641854E-5,8.14102058654018E-5,8.2812112065706E-5,
8.70178306666183E-5,0.000116081955658528,0.000130526745999927,0.000162394111022038,
0.000174035661333236,0.000213138396956903,0.000256116935431176,0.000302406662852235,
0.000348071322666485),.UNSPECIFIED.);
#4558=B_SPLINE_CURVE_WITH_KNOTS('',3,(#188963,#188964,#188965,#188966,#188967,
#188968,#188969,#188970,#188971,#188972,#188973,#188974,#188975,#188976,
#188977,#188978,#188979,#188980,#188981,#188982,#188983,#188984,#188985,
#188986,#188987,#188988,#188989,#188990,#188991,#188992,#188993,#188994,
#188995,#188996,#188997,#188998,#188999,#189000,#189001,#189002,#189003,
#189004,#189005,#189006,#189007,#189008,#189009,#189010,#189011,#189012,
#189013,#189014),.UNSPECIFIED.,.F.,.F.,(4,3,3,3,3,3,3,3,3,3,3,3,3,3,3,3,
3,4),(0.,4.29652152157141E-5,8.44519107528248E-5,0.000123669830864298,0.000159788877357386,
0.000170558847912639,0.000181218775907179,0.000181960046452421,0.000214460062643711,
0.000244755726198599,0.000255838271868953,0.000258503253867588,0.000261084955178765,
0.000289370476647698,0.000301101325502016,0.000321109510663641,0.000331113603244454,
0.000341117695825267),.UNSPECIFIED.);
#4559=B_SPLINE_CURVE_WITH_KNOTS('',3,(#189016,#189017,#189018,#189019,#189020,
#189021,#189022,#189023,#189024,#189025,#189026,#189027,#189028,#189029,
#189030,#189031,#189032,#189033,#189034,#189035,#189036,#189037,#189038,
#189039,#189040,#189041,#189042,#189043,#189044,#189045,#189046,#189047,
#189048,#189049,#189050,#189051,#189052,#189053,#189054,#189055,#189056,
#189057,#189058,#189059,#189060,#189061,#189062,#189063,#189064,#189065,
#189066,#189067),.UNSPECIFIED.,.F.,.F.,(4,3,3,3,3,3,3,3,3,3,3,3,3,3,3,3,
3,4),(0.,4.30706237863024E-5,8.47417087684952E-5,0.000124159989204232,0.000160467076288062,
0.000170998382116688,0.000182414994733777,0.000213747977645863,0.000242415955901826,
0.000256497573175038,0.000259169422895611,0.000261757777312417,0.000289965130404822,
0.000301877270772903,0.000321937017503145,0.000326951954185706,0.000334474359209547,
0.000341996764233388),.UNSPECIFIED.);
#4560=B_SPLINE_CURVE_WITH_KNOTS('',3,(#189068,#189069,#189070,#189071,#189072,
#189073,#189074,#189075,#189076,#189077,#189078,#189079,#189080,#189081,
#189082,#189083,#189084,#189085,#189086,#189087,#189088,#189089,#189090,
#189091,#189092,#189093,#189094,#189095,#189096,#189097,#189098,#189099,
#189100,#189101,#189102,#189103,#189104,#189105,#189106,#189107,#189108,
#189109,#189110,#189111,#189112,#189113,#189114,#189115,#189116,#189117,
#189118,#189119),.UNSPECIFIED.,.F.,.F.,(4,3,3,3,3,3,3,3,3,3,3,3,3,3,3,3,
3,4),(0.,2.58457451673335E-5,4.25394446194833E-5,6.46659869686626E-5,7.57292581432522E-5,
8.12608937305471E-5,8.26438026273708E-5,8.67925293178419E-5,0.000116015624427352,
0.000130188793976763,0.000151886926306223,0.000161963651211264,0.000162735992470954,
0.000173585058635684,0.000212487880460423,0.000255238173509651,0.000301397761141473,
0.000347170117271379),.UNSPECIFIED.);
#4561=B_SPLINE_CURVE_WITH_KNOTS('',3,(#189121,#189122,#189123,#189124,#189125,
#189126,#189127,#189128,#189129,#189130,#189131,#189132,#189133,#189134,
#189135,#189136,#189137,#189138,#189139,#189140,#189141,#189142,#189143,
#189144,#189145,#189146,#189147,#189148,#189149,#189150,#189151,#189152,
#189153,#189154,#189155,#189156,#189157,#189158,#189159,#189160,#189161,
#189162,#189163,#189164,#189165,#189166),.UNSPECIFIED.,.F.,.F.,(4,3,3,3,
3,3,3,3,3,3,3,3,3,3,3,4),(0.,2.57218161990161E-5,4.21568322567036E-5,6.45873314616669E-5,
7.58025810641486E-5,8.14102058653895E-5,8.28121120656997E-5,8.70178306666303E-5,
0.000116081955657631,0.000130526745999942,0.000162394111022068,0.000174035661333253,
0.000213138396958698,0.00025611693543461,0.000302406662857067,0.000348071322666475),
 .UNSPECIFIED.);
#4562=B_SPLINE_CURVE_WITH_KNOTS('',3,(#189167,#189168,#189169,#189170,#189171,
#189172,#189173,#189174,#189175,#189176,#189177,#189178,#189179,#189180,
#189181,#189182,#189183,#189184,#189185,#189186,#189187,#189188,#189189,
#189190,#189191,#189192,#189193,#189194,#189195,#189196,#189197,#189198,
#189199,#189200,#189201,#189202,#189203,#189204,#189205,#189206,#189207,
#189208,#189209,#189210,#189211,#189212,#189213,#189214,#189215,#189216,
#189217,#189218),.UNSPECIFIED.,.F.,.F.,(4,3,3,3,3,3,3,3,3,3,3,3,3,3,3,3,
3,4),(0.,4.29652152166112E-5,8.44519107541718E-5,0.000123669830865709,0.00015978887735854,
0.00017055884791262,0.000181218775907161,0.000181960046452391,0.000214460062643901,
0.000244755726199277,0.000255838271868943,0.000258503253867579,0.000261084955178756,
0.000289370476647179,0.000301101325502011,0.000321109510663639,0.000331113603244453,
0.000341117695825267),.UNSPECIFIED.);
#4563=B_SPLINE_CURVE_WITH_KNOTS('',3,(#189220,#189221,#189222,#189223,#189224,
#189225,#189226,#189227,#189228,#189229,#189230,#189231,#189232,#189233,
#189234,#189235,#189236,#189237,#189238,#189239,#189240,#189241,#189242,
#189243,#189244,#189245,#189246,#189247,#189248,#189249,#189250,#189251,
#189252,#189253,#189254,#189255,#189256,#189257,#189258,#189259,#189260,
#189261,#189262,#189263,#189264,#189265,#189266,#189267,#189268,#189269,
#189270,#189271),.UNSPECIFIED.,.F.,.F.,(4,3,3,3,3,3,3,3,3,3,3,3,3,3,3,3,
3,4),(0.,4.3070623786285E-5,8.47417087683859E-5,0.000124159989203828,0.000160467076287352,
0.000170998382116686,0.000182414994733794,0.00021374797764586,0.000242415955901968,
0.000256497573175035,0.000259169422895608,0.000261757777312414,0.000289965130404094,
0.000301877270772899,0.000321937017503141,0.000326951954185702,0.000334474359209543,
0.000341996764233384),.UNSPECIFIED.);
#4564=B_SPLINE_CURVE_WITH_KNOTS('',3,(#189272,#189273,#189274,#189275,#189276,
#189277,#189278,#189279,#189280,#189281,#189282,#189283,#189284,#189285,
#189286,#189287,#189288,#189289,#189290,#189291,#189292,#189293,#189294,
#189295,#189296,#189297,#189298,#189299,#189300,#189301,#189302,#189303,
#189304,#189305,#189306,#189307,#189308,#189309,#189310,#189311,#189312,
#189313,#189314,#189315,#189316,#189317,#189318,#189319,#189320,#189321,
#189322,#189323),.UNSPECIFIED.,.F.,.F.,(4,3,3,3,3,3,3,3,3,3,3,3,3,3,3,3,
3,4),(0.,2.58457451685046E-5,4.25394446195917E-5,6.46659869687147E-5,7.57292581432762E-5,
8.12608937305569E-5,8.26438026273771E-5,8.67925293178377E-5,0.000116015624427896,
0.000130188793976757,0.000151886926306216,0.000161963651211271,0.000162735992470946,
0.000173585058635675,0.000212487880458822,0.000255238173506331,0.000301397761136081,
0.000347170117271363),.UNSPECIFIED.);
#4565=B_SPLINE_CURVE_WITH_KNOTS('',3,(#189325,#189326,#189327,#189328,#189329,
#189330,#189331,#189332,#189333,#189334,#189335,#189336,#189337,#189338,
#189339,#189340,#189341,#189342,#189343,#189344,#189345,#189346,#189347,
#189348,#189349,#189350,#189351,#189352,#189353,#189354,#189355,#189356,
#189357,#189358,#189359,#189360,#189361,#189362,#189363,#189364,#189365,
#189366,#189367,#189368,#189369,#189370),.UNSPECIFIED.,.F.,.F.,(4,3,3,3,
3,3,3,3,3,3,3,3,3,3,3,4),(0.,2.57218162002362E-5,4.21568322566886E-5,6.45873314616546E-5,
7.58025810641376E-5,8.14102058653791E-5,8.28121120656895E-5,8.70178306666206E-5,
0.000116081955657556,0.000130526745999931,0.000162394111022038,0.000174035661333241,
0.000213138396957546,0.000256116935432267,0.000302406662853359,0.000348071322666503),
 .UNSPECIFIED.);
#4566=B_SPLINE_CURVE_WITH_KNOTS('',3,(#189371,#189372,#189373,#189374,#189375,
#189376,#189377,#189378,#189379,#189380,#189381,#189382,#189383,#189384,
#189385,#189386,#189387,#189388,#189389,#189390,#189391,#189392,#189393,
#189394,#189395,#189396,#189397,#189398,#189399,#189400,#189401,#189402,
#189403,#189404,#189405,#189406,#189407,#189408,#189409,#189410,#189411,
#189412,#189413,#189414,#189415,#189416,#189417,#189418,#189419,#189420,
#189421,#189422),.UNSPECIFIED.,.F.,.F.,(4,3,3,3,3,3,3,3,3,3,3,3,3,3,3,3,
3,4),(0.,4.29652152209911E-5,8.44519107613256E-5,0.000123669830874747,0.00015978887736901,
0.000170558847912628,0.000181218775907169,0.000181960046452397,0.000214460062644086,
0.000244755726200129,0.00025583827186895,0.000258503253867585,0.000261084955178762,
0.000289370476647124,0.000301101325502017,0.000321109510663644,0.000331113603244457,
0.000341117695825271),.UNSPECIFIED.);
#4567=B_SPLINE_CURVE_WITH_KNOTS('',3,(#189424,#189425,#189426,#189427,#189428,
#189429,#189430,#189431,#189432,#189433,#189434,#189435,#189436,#189437,
#189438,#189439,#189440,#189441,#189442,#189443,#189444,#189445,#189446,
#189447,#189448,#189449,#189450,#189451,#189452,#189453,#189454,#189455,
#189456,#189457,#189458,#189459,#189460,#189461,#189462,#189463,#189464,
#189465,#189466,#189467,#189468,#189469,#189470,#189471,#189472,#189473,
#189474,#189475),.UNSPECIFIED.,.F.,.F.,(4,3,3,3,3,3,3,3,3,3,3,3,3,3,3,3,
3,4),(0.,4.3070623786733E-5,8.47417087690687E-5,0.000124159989204553,0.000160467076288069,
0.000170998382116701,0.000182414994733781,0.000213747977645875,0.00024241595590332,
0.000256497573175049,0.000259169422895622,0.000261757777312428,0.000289965130403643,
0.000301877270772912,0.000321937017503154,0.000326951954185715,0.000334474359209555,
0.000341996764233396),.UNSPECIFIED.);
#4568=B_SPLINE_CURVE_WITH_KNOTS('',3,(#189476,#189477,#189478,#189479,#189480,
#189481,#189482,#189483,#189484,#189485,#189486,#189487,#189488,#189489,
#189490,#189491,#189492,#189493,#189494,#189495,#189496,#189497,#189498,
#189499,#189500,#189501,#189502,#189503,#189504,#189505,#189506,#189507,
#189508,#189509,#189510,#189511,#189512,#189513,#189514,#189515,#189516,
#189517,#189518,#189519,#189520,#189521,#189522,#189523,#189524,#189525,
#189526,#189527),.UNSPECIFIED.,.F.,.F.,(4,3,3,3,3,3,3,3,3,3,3,3,3,3,3,3,
3,4),(0.,2.5845745166866E-5,4.25394446195452E-5,6.46659869686944E-5,7.5729258143269E-5,
8.12608937305563E-5,8.26438026273781E-5,8.67925293178436E-5,0.000116015624427498,
0.000130188793976765,0.000151886926306226,0.000161963651211271,0.000162735992470957,
0.000173585058635687,0.000212487880461328,0.000255238173512605,0.000301397761148938,
0.00034717011727138),.UNSPECIFIED.);
#4569=B_SPLINE_CURVE_WITH_KNOTS('',3,(#189529,#189530,#189531,#189532,#189533,
#189534,#189535,#189536,#189537,#189538,#189539,#189540,#189541,#189542,
#189543,#189544,#189545,#189546,#189547,#189548,#189549,#189550,#189551,
#189552,#189553,#189554,#189555,#189556,#189557,#189558,#189559,#189560,
#189561,#189562,#189563,#189564,#189565,#189566,#189567,#189568,#189569,
#189570,#189571,#189572,#189573,#189574),.UNSPECIFIED.,.F.,.F.,(4,3,3,3,
3,3,3,3,3,3,3,3,3,3,3,4),(0.,2.57218161987294E-5,4.21568322567358E-5,6.45873314616753E-5,
7.5802581064145E-5,8.14102058653799E-5,8.28121120656886E-5,8.70178306666148E-5,
0.000116081955659026,0.000130526745999922,0.000162394111022043,0.00017403566133323,
0.000213138396960531,0.000256116935438422,0.000302406662863451,0.000348071322666455),
 .UNSPECIFIED.);
#4570=B_SPLINE_CURVE_WITH_KNOTS('',3,(#189575,#189576,#189577,#189578,#189579,
#189580,#189581,#189582,#189583,#189584,#189585,#189586,#189587,#189588,
#189589,#189590,#189591,#189592,#189593,#189594,#189595,#189596,#189597,
#189598,#189599,#189600,#189601,#189602,#189603,#189604,#189605,#189606,
#189607,#189608,#189609,#189610,#189611,#189612,#189613,#189614,#189615,
#189616,#189617,#189618,#189619,#189620,#189621,#189622,#189623,#189624,
#189625,#189626),.UNSPECIFIED.,.F.,.F.,(4,3,3,3,3,3,3,3,3,3,3,3,3,3,3,3,
3,4),(0.,4.29652152174181E-5,8.44519107551507E-5,0.00012366983086629,0.000159788877358252,
0.000170558847912638,0.000181218775907176,0.000181960046452432,0.000214460062643755,
0.000244755726198294,0.000255838271868943,0.000258503253867577,0.000261084955178754,
0.000289370476647915,0.000301101325502001,0.000321109510663624,0.000331113603244436,
0.000341117695825248),.UNSPECIFIED.);
#4571=B_SPLINE_CURVE_WITH_KNOTS('',3,(#189628,#189629,#189630,#189631,#189632,
#189633,#189634,#189635,#189636,#189637,#189638,#189639,#189640,#189641,
#189642,#189643,#189644,#189645,#189646,#189647,#189648,#189649,#189650,
#189651,#189652,#189653,#189654,#189655,#189656,#189657,#189658,#189659,
#189660,#189661,#189662,#189663,#189664,#189665,#189666,#189667,#189668,
#189669,#189670,#189671,#189672,#189673,#189674,#189675,#189676,#189677,
#189678,#189679),.UNSPECIFIED.,.F.,.F.,(4,3,3,3,3,3,3,3,3,3,3,3,3,3,3,3,
3,4),(0.,4.30706237872049E-5,8.47417087702058E-5,0.000124159989206704,0.000160467076291566,
0.000170998382116693,0.000182414994733776,0.000213747977645866,0.000242415955902374,
0.000256497573175039,0.000259169422895612,0.000261757777312417,0.000289965130404078,
0.000301877270772901,0.000321937017503142,0.000326951954185703,0.000334474359209543,
0.000341996764233384),.UNSPECIFIED.);
#4572=B_SPLINE_CURVE_WITH_KNOTS('',3,(#189680,#189681,#189682,#189683,#189684,
#189685,#189686,#189687,#189688,#189689,#189690,#189691,#189692,#189693,
#189694,#189695,#189696,#189697,#189698,#189699,#189700,#189701,#189702,
#189703,#189704,#189705,#189706,#189707,#189708,#189709,#189710,#189711,
#189712,#189713,#189714,#189715,#189716,#189717,#189718,#189719,#189720,
#189721,#189722,#189723,#189724,#189725,#189726,#189727,#189728,#189729,
#189730,#189731),.UNSPECIFIED.,.F.,.F.,(4,3,3,3,3,3,3,3,3,3,3,3,3,3,3,3,
3,4),(3.46944695195361E-18,2.58457451679455E-5,4.25394446195489E-5,6.46659869686949E-5,
7.57292581432678E-5,8.12608937305543E-5,8.2643802627376E-5,8.67925293178408E-5,
0.000116015624426877,0.000130188793976759,0.000151886926306219,0.000161963651211276,
0.000162735992470949,0.000173585058635678,0.000212487880458077,0.000255238173504525,
0.000301397761132519,0.000347170117271368),.UNSPECIFIED.);
#4573=B_SPLINE_CURVE_WITH_KNOTS('',3,(#189733,#189734,#189735,#189736,#189737,
#189738,#189739,#189740,#189741,#189742,#189743,#189744,#189745,#189746,
#189747,#189748,#189749,#189750,#189751,#189752,#189753,#189754,#189755,
#189756,#189757,#189758,#189759,#189760,#189761,#189762,#189763,#189764,
#189765,#189766,#189767,#189768,#189769,#189770,#189771,#189772,#189773,
#189774,#189775,#189776,#189777,#189778),.UNSPECIFIED.,.F.,.F.,(4,3,3,3,
3,3,3,3,3,3,3,3,3,3,3,4),(3.46944695195361E-18,2.57218162010662E-5,4.21568322569032E-5,
6.45873314617582E-5,7.58025810641856E-5,8.14102058653994E-5,8.28121120657028E-5,
8.70178306666131E-5,0.000116081955659514,0.000130526745999918,0.00016239411102203,
0.000174035661333223,0.000213138396958463,0.000256116935434209,0.000302406662856632,
0.000348071322666446),.UNSPECIFIED.);
#4574=B_SPLINE_CURVE_WITH_KNOTS('',3,(#189779,#189780,#189781,#189782,#189783,
#189784,#189785,#189786,#189787,#189788,#189789,#189790,#189791,#189792,
#189793,#189794,#189795,#189796,#189797,#189798,#189799,#189800,#189801,
#189802,#189803,#189804,#189805,#189806,#189807,#189808,#189809,#189810,
#189811,#189812,#189813,#189814,#189815,#189816,#189817,#189818,#189819,
#189820,#189821,#189822,#189823,#189824,#189825,#189826,#189827,#189828,
#189829,#189830),.UNSPECIFIED.,.F.,.F.,(4,3,3,3,3,3,3,3,3,3,3,3,3,3,3,3,
3,4),(0.,4.2965215219084E-5,8.44519107582157E-5,0.000123669830870834,0.000159788877364523,
0.000170558847912632,0.000181218775907171,0.000181960046452412,0.000214460062643453,
0.000244755726197965,0.000255838271868945,0.000258503253867579,0.000261084955178757,
0.000289370476647428,0.000301101325502007,0.000321109510663632,0.000331113603244445,
0.000341117695825257),.UNSPECIFIED.);
#4575=B_SPLINE_CURVE_WITH_KNOTS('',3,(#189832,#189833,#189834,#189835,#189836,
#189837,#189838,#189839,#189840,#189841,#189842,#189843,#189844,#189845,
#189846,#189847,#189848,#189849,#189850,#189851,#189852,#189853,#189854,
#189855,#189856,#189857,#189858,#189859,#189860,#189861,#189862,#189863,
#189864,#189865,#189866,#189867,#189868,#189869,#189870,#189871,#189872,
#189873,#189874,#189875,#189876,#189877,#189878,#189879,#189880,#189881,
#189882,#189883),.UNSPECIFIED.,.F.,.F.,(4,3,3,3,3,3,3,3,3,3,3,3,3,3,3,3,
3,4),(0.,4.30706237872751E-5,8.47417087704076E-5,0.000124159989207045,0.000160467076291976,
0.000170998382116688,0.000182414994733785,0.000213747977645864,0.000242415955904398,
0.000256497573175039,0.000259169422895612,0.000261757777312418,0.000289965130402912,
0.000301877270772903,0.000321937017503146,0.000326951954185707,0.000334474359209548,
0.000341996764233389),.UNSPECIFIED.);
#4576=B_SPLINE_CURVE_WITH_KNOTS('',3,(#189884,#189885,#189886,#189887,#189888,
#189889,#189890,#189891,#189892,#189893,#189894,#189895,#189896,#189897,
#189898,#189899,#189900,#189901,#189902,#189903,#189904,#189905,#189906,
#189907,#189908,#189909,#189910,#189911,#189912,#189913,#189914,#189915,
#189916,#189917,#189918,#189919,#189920,#189921,#189922,#189923,#189924,
#189925,#189926,#189927,#189928,#189929,#189930,#189931,#189932,#189933,
#189934,#189935),.UNSPECIFIED.,.F.,.F.,(4,3,3,3,3,3,3,3,3,3,3,3,3,3,3,3,
3,4),(0.,2.58457451679569E-5,4.25394446195776E-5,6.46659869687099E-5,7.5729258143276E-5,
8.12608937305591E-5,8.26438026273799E-5,8.67925293178422E-5,0.000116015624427706,
0.000130188793976763,0.000151886926306224,0.000161963651211281,0.000162735992470954,
0.000173585058635684,0.000212487880460481,0.000255238173510222,0.000301397761143518,
0.000347170117271362),.UNSPECIFIED.);
#4577=B_SPLINE_CURVE_WITH_KNOTS('',3,(#189937,#189938,#189939,#189940,#189941,
#189942,#189943,#189944,#189945,#189946,#189947,#189948,#189949,#189950,
#189951,#189952,#189953,#189954,#189955,#189956,#189957,#189958,#189959,
#189960,#189961,#189962,#189963,#189964,#189965,#189966,#189967,#189968,
#189969,#189970,#189971,#189972,#189973,#189974,#189975,#189976,#189977,
#189978,#189979,#189980,#189981,#189982),.UNSPECIFIED.,.F.,.F.,(4,3,3,3,
3,3,3,3,3,3,3,3,3,3,3,4),(0.,2.57218161989729E-5,4.21568322568806E-5,6.45873314617506E-5,
7.58025810641856E-5,8.14102058654031E-5,8.28121120657075E-5,8.70178306666206E-5,
0.000116081955658818,0.000130526745999931,0.000162394111022037,0.000174035661333241,
0.000213138396956396,0.000256116935430151,0.000302406662850685,0.000348071322666478),
 .UNSPECIFIED.);
#4578=B_SPLINE_CURVE_WITH_KNOTS('',3,(#189983,#189984,#189985,#189986,#189987,
#189988,#189989,#189990,#189991,#189992,#189993,#189994,#189995,#189996,
#189997,#189998,#189999,#190000,#190001,#190002,#190003,#190004,#190005,
#190006,#190007,#190008,#190009,#190010,#190011,#190012,#190013,#190014,
#190015,#190016,#190017,#190018,#190019,#190020,#190021,#190022,#190023,
#190024,#190025,#190026,#190027,#190028,#190029,#190030,#190031,#190032,
#190033,#190034),.UNSPECIFIED.,.F.,.F.,(4,3,3,3,3,3,3,3,3,3,3,3,3,3,3,3,
3,4),(0.,4.29652152136548E-5,8.44519107495283E-5,0.000123669830860329,0.000159788877352937,
0.000170558847912617,0.000181218775907158,0.000181960046452403,0.000214460062643498,
0.000244755726198013,0.00025583827186894,0.000258503253867575,0.000261084955178752,
0.000289370476647941,0.000301101325502007,0.000321109510663635,0.000331113603244448,
0.000341117695825262),.UNSPECIFIED.);
#4579=B_SPLINE_CURVE_WITH_KNOTS('',3,(#190036,#190037,#190038,#190039,#190040,
#190041,#190042,#190043,#190044,#190045,#190046,#190047,#190048,#190049,
#190050,#190051,#190052,#190053,#190054,#190055,#190056,#190057,#190058,
#190059,#190060,#190061,#190062,#190063,#190064,#190065,#190066,#190067,
#190068,#190069,#190070,#190071,#190072,#190073,#190074,#190075,#190076,
#190077,#190078,#190079,#190080,#190081,#190082,#190083,#190084,#190085,
#190086,#190087),.UNSPECIFIED.,.F.,.F.,(4,3,3,3,3,3,3,3,3,3,3,3,3,3,3,3,
3,4),(0.,4.30706237876541E-5,8.47417087708983E-5,0.000124159989207408,0.00016046707629211,
0.000170998382116697,0.000182414994733759,0.00021374797764587,0.000242415955902421,
0.000256497573175043,0.000259169422895616,0.000261757777312422,0.000289965130404187,
0.000301877270772906,0.000321937017503147,0.000326951954185708,0.000334474359209549,
0.000341996764233389),.UNSPECIFIED.);
#4580=B_SPLINE_CURVE_WITH_KNOTS('',3,(#190088,#190089,#190090,#190091,#190092,
#190093,#190094,#190095,#190096,#190097,#190098,#190099,#190100,#190101,
#190102,#190103,#190104,#190105,#190106,#190107,#190108,#190109,#190110,
#190111,#190112,#190113,#190114,#190115,#190116,#190117,#190118,#190119,
#190120,#190121,#190122,#190123,#190124,#190125,#190126,#190127,#190128,
#190129,#190130,#190131,#190132,#190133,#190134,#190135,#190136,#190137,
#190138,#190139),.UNSPECIFIED.,.F.,.F.,(4,3,3,3,3,3,3,3,3,3,3,3,3,3,3,3,
3,4),(0.,2.58457451677454E-5,4.25394446195769E-5,6.4665986968705E-5,7.5729258143269E-5,
8.1260893730551E-5,8.26438026273715E-5,8.6792529317833E-5,0.000116015624427558,
0.00013018879397675,0.000151886926306208,0.000161963651211251,0.000162735992470937,
0.000173585058635666,0.000212487880460707,0.00025523817351233,0.00030139776115075,
0.000347170117271366),.UNSPECIFIED.);
#4581=B_SPLINE_CURVE_WITH_KNOTS('',3,(#190141,#190142,#190143,#190144,#190145,
#190146,#190147,#190148,#190149,#190150,#190151,#190152,#190153,#190154,
#190155,#190156,#190157,#190158,#190159,#190160,#190161,#190162,#190163,
#190164,#190165,#190166,#190167,#190168,#190169,#190170,#190171,#190172,
#190173,#190174,#190175,#190176,#190177,#190178,#190179,#190180,#190181,
#190182,#190183,#190184,#190185,#190186),.UNSPECIFIED.,.F.,.F.,(4,3,3,3,
3,3,3,3,3,3,3,3,3,3,3,4),(0.,2.57218162002616E-5,4.21568322567789E-5,6.45873314616992E-5,
7.58025810641594E-5,8.14102058653895E-5,8.2812112065697E-5,8.70178306666196E-5,
0.000116081955657916,0.000130526745999929,0.000162394111022025,0.000174035661333239,
0.000213138396954118,0.000256116935425588,0.000302406662843531,0.000348071322666471),
 .UNSPECIFIED.);
#4582=B_SPLINE_CURVE_WITH_KNOTS('',3,(#190187,#190188,#190189,#190190,#190191,
#190192,#190193,#190194,#190195,#190196,#190197,#190198,#190199,#190200,
#190201,#190202,#190203,#190204,#190205,#190206,#190207,#190208,#190209,
#190210,#190211,#190212,#190213,#190214,#190215,#190216,#190217,#190218,
#190219,#190220,#190221,#190222,#190223,#190224,#190225,#190226,#190227,
#190228,#190229,#190230,#190231,#190232,#190233,#190234,#190235,#190236,
#190237,#190238),.UNSPECIFIED.,.F.,.F.,(4,3,3,3,3,3,3,3,3,3,3,3,3,3,3,3,
3,4),(0.,4.29652152132578E-5,8.44519107492023E-5,0.000123669830860594,0.000159788877354395,
0.000170558847912621,0.00018121877590716,0.000181960046452396,0.000214460062643361,
0.000244755726197735,0.000255838271868937,0.000258503253867572,0.00026108495517875,
0.00028937047664799,0.000301101325502002,0.000321109510663628,0.000331113603244441,
0.000341117695825254),.UNSPECIFIED.);
#4583=B_SPLINE_CURVE_WITH_KNOTS('',3,(#190240,#190241,#190242,#190243,#190244,
#190245,#190246,#190247,#190248,#190249,#190250,#190251,#190252,#190253,
#190254,#190255,#190256,#190257,#190258,#190259,#190260,#190261,#190262,
#190263,#190264,#190265,#190266,#190267,#190268,#190269,#190270,#190271,
#190272,#190273,#190274,#190275,#190276,#190277,#190278,#190279,#190280,
#190281,#190282,#190283,#190284,#190285,#190286,#190287,#190288,#190289,
#190290,#190291),.UNSPECIFIED.,.F.,.F.,(4,3,3,3,3,3,3,3,3,3,3,3,3,3,3,3,
3,4),(0.,4.30706237885874E-5,8.47417087727397E-5,0.000124159989210242,0.000160467076296224,
0.000170998382116709,0.000182414994733818,0.000213747977645879,0.000242415955903209,
0.000256497573175049,0.000259169422895622,0.000261757777312427,0.00028996513040331,
0.000301877270772908,0.000321937017503148,0.000326951954185708,0.000334474359209549,
0.000341996764233389),.UNSPECIFIED.);
#4584=B_SPLINE_CURVE_WITH_KNOTS('',3,(#190292,#190293,#190294,#190295,#190296,
#190297,#190298,#190299,#190300,#190301,#190302,#190303,#190304,#190305,
#190306,#190307,#190308,#190309,#190310,#190311,#190312,#190313,#190314,
#190315,#190316,#190317,#190318,#190319,#190320,#190321,#190322,#190323,
#190324,#190325,#190326,#190327,#190328,#190329,#190330,#190331,#190332,
#190333,#190334,#190335,#190336,#190337,#190338,#190339,#190340,#190341,
#190342,#190343),.UNSPECIFIED.,.F.,.F.,(4,3,3,3,3,3,3,3,3,3,3,3,3,3,3,3,
3,4),(0.,2.58457451690894E-5,4.25394446196487E-5,6.46659869687494E-5,7.57292581432998E-5,
8.1260893730575E-5,8.26438026273938E-5,8.67925293178501E-5,0.000116015624428787,
0.000130188793976775,0.000151886926306238,0.000161963651211307,0.000162735992470969,
0.0001735850586357,0.000212487880461016,0.000255238173513134,0.00030139776115256,
0.000347170117271371),.UNSPECIFIED.);
#4585=B_SPLINE_CURVE_WITH_KNOTS('',3,(#190345,#190346,#190347,#190348,#190349,
#190350,#190351,#190352,#190353,#190354,#190355,#190356,#190357,#190358,
#190359,#190360,#190361,#190362,#190363,#190364,#190365,#190366,#190367,
#190368,#190369,#190370,#190371,#190372,#190373,#190374,#190375,#190376,
#190377,#190378,#190379,#190380,#190381,#190382,#190383,#190384,#190385,
#190386,#190387,#190388,#190389,#190390),.UNSPECIFIED.,.F.,.F.,(4,3,3,3,
3,3,3,3,3,3,3,3,3,3,3,4),(0.,2.57218161979397E-5,4.21568322566978E-5,6.45873314616655E-5,
7.58025810641494E-5,8.14102058653913E-5,8.28121120657018E-5,8.70178306666332E-5,
0.000116081955659105,0.00013052674599995,0.000162394111022055,0.000174035661333266,
0.000213138396958747,0.000256116935434786,0.000302406662857728,0.0003480713226665),
 .UNSPECIFIED.);
#4586=B_SPLINE_CURVE_WITH_KNOTS('',3,(#190391,#190392,#190393,#190394,#190395,
#190396,#190397,#190398,#190399,#190400,#190401,#190402,#190403,#190404,
#190405,#190406,#190407,#190408,#190409,#190410,#190411,#190412,#190413,
#190414,#190415,#190416,#190417,#190418,#190419,#190420,#190421,#190422,
#190423,#190424,#190425,#190426,#190427,#190428,#190429,#190430,#190431,
#190432,#190433,#190434,#190435,#190436,#190437,#190438,#190439,#190440,
#190441,#190442),.UNSPECIFIED.,.F.,.F.,(4,3,3,3,3,3,3,3,3,3,3,3,3,3,3,3,
3,4),(0.,4.29652152110204E-5,8.44519107444466E-5,0.00012366983085245,0.000159788877341661,
0.000170558847912638,0.000181218775907178,0.000181960046452416,0.000214460062642894,
0.00024475572619666,0.000255838271868955,0.00025850325386759,0.000261084955178768,
0.000289370476650761,0.00030110132550202,0.000321109510663647,0.00033111360324446,
0.000341117695825273),.UNSPECIFIED.);
#4587=B_SPLINE_CURVE_WITH_KNOTS('',3,(#190444,#190445,#190446,#190447,#190448,
#190449,#190450,#190451,#190452,#190453,#190454,#190455,#190456,#190457,
#190458,#190459,#190460,#190461,#190462,#190463,#190464,#190465,#190466,
#190467,#190468,#190469,#190470,#190471,#190472,#190473,#190474,#190475,
#190476,#190477,#190478,#190479,#190480,#190481,#190482,#190483,#190484,
#190485,#190486,#190487,#190488,#190489,#190490,#190491,#190492,#190493,
#190494,#190495),.UNSPECIFIED.,.F.,.F.,(4,3,3,3,3,3,3,3,3,3,3,3,3,3,3,3,
3,4),(0.,4.30706237889129E-5,8.47417087731407E-5,0.000124159989210559,0.000160467076296243,
0.000170998382116688,0.00018241499473377,0.000213747977645864,0.000242415955903622,
0.000256497573175039,0.000259169422895612,0.000261757777312418,0.000289965130404044,
0.000301877270772903,0.000321937017503146,0.000326951954185707,0.000334474359209548,
0.000341996764233389),.UNSPECIFIED.);
#4588=B_SPLINE_CURVE_WITH_KNOTS('',3,(#190496,#190497,#190498,#190499,#190500,
#190501,#190502,#190503,#190504,#190505,#190506,#190507,#190508,#190509,
#190510,#190511,#190512,#190513,#190514,#190515,#190516,#190517,#190518,
#190519,#190520,#190521,#190522,#190523,#190524,#190525,#190526,#190527,
#190528,#190529,#190530,#190531,#190532,#190533,#190534,#190535,#190536,
#190537,#190538,#190539,#190540,#190541,#190542,#190543,#190544,#190545,
#190546,#190547),.UNSPECIFIED.,.F.,.F.,(4,3,3,3,3,3,3,3,3,3,3,3,3,3,3,3,
3,4),(0.,2.58457451665418E-5,4.25394446196923E-5,6.46659869687673E-5,7.57292581433048E-5,
8.12608937305736E-5,8.26438026273908E-5,8.67925293178423E-5,0.000116015624427747,
0.000130188793976764,0.000151886926306224,0.000161963651211288,0.000162735992470954,
0.000173585058635685,0.000212487880459422,0.000255238173507843,0.00030139776113927,
0.000347170117271382),.UNSPECIFIED.);
#4589=B_SPLINE_CURVE_WITH_KNOTS('',3,(#190549,#190550,#190551,#190552,#190553,
#190554,#190555,#190556,#190557,#190558,#190559,#190560,#190561,#190562,
#190563,#190564,#190565,#190566,#190567,#190568,#190569,#190570,#190571,
#190572,#190573,#190574,#190575,#190576,#190577,#190578,#190579,#190580,
#190581,#190582,#190583,#190584,#190585,#190586,#190587,#190588,#190589,
#190590,#190591,#190592,#190593,#190594),.UNSPECIFIED.,.F.,.F.,(4,3,3,3,
3,3,3,3,3,3,3,3,3,3,3,4),(0.,2.57218161992769E-5,4.21568322568503E-5,6.45873314617301E-5,
7.58025810641699E-5,8.14102058653899E-5,8.28121120656949E-5,8.70178306666098E-5,
0.000116081955658396,0.000130526745999915,0.00016239411102202,0.00017403566133322,
0.00021313839696102,0.000256116935439445,0.000302406662865238,0.000348071322666453),
 .UNSPECIFIED.);
#4590=B_SPLINE_CURVE_WITH_KNOTS('',3,(#190595,#190596,#190597,#190598,#190599,
#190600,#190601,#190602,#190603,#190604,#190605,#190606,#190607,#190608,
#190609,#190610,#190611,#190612,#190613,#190614,#190615,#190616,#190617,
#190618,#190619,#190620,#190621,#190622,#190623,#190624,#190625,#190626,
#190627,#190628,#190629,#190630,#190631,#190632,#190633,#190634,#190635,
#190636,#190637,#190638,#190639,#190640,#190641,#190642,#190643,#190644,
#190645,#190646),.UNSPECIFIED.,.F.,.F.,(4,3,3,3,3,3,3,3,3,3,3,3,3,3,3,3,
3,4),(0.,4.29652152249339E-5,8.44519107677232E-5,0.000123669830882601,0.000159788877377764,
0.000170558847912626,0.000181218775907166,0.000181960046452394,0.000214460062643825,
0.000244755726198773,0.000255838271868946,0.000258503253867581,0.000261084955178759,
0.000289370476647345,0.000301101325502013,0.000321109510663639,0.000331113603244453,
0.000341117695825266),.UNSPECIFIED.);
#4591=B_SPLINE_CURVE_WITH_KNOTS('',3,(#190648,#190649,#190650,#190651,#190652,
#190653,#190654,#190655,#190656,#190657,#190658,#190659,#190660,#190661,
#190662,#190663,#190664,#190665,#190666,#190667,#190668,#190669,#190670,
#190671,#190672,#190673,#190674,#190675,#190676,#190677,#190678,#190679,
#190680,#190681,#190682,#190683,#190684,#190685,#190686,#190687,#190688,
#190689,#190690,#190691,#190692,#190693,#190694,#190695,#190696,#190697,
#190698,#190699),.UNSPECIFIED.,.F.,.F.,(4,3,3,3,3,3,3,3,3,3,3,3,3,3,3,3,
3,4),(0.,4.30706237852771E-5,8.47417087665961E-5,0.000124159989201271,0.000160467076283982,
0.000170998382116692,0.000182414994733772,0.000213747977645867,0.000242415955903141,
0.000256497573175042,0.000259169422895616,0.000261757777312421,0.000289965130404113,
0.000301877270772907,0.000321937017503149,0.00032695195418571,0.000334474359209551,
0.000341996764233392),.UNSPECIFIED.);
#4592=B_SPLINE_CURVE_WITH_KNOTS('',3,(#190700,#190701,#190702,#190703,#190704,
#190705,#190706,#190707,#190708,#190709,#190710,#190711,#190712,#190713,
#190714,#190715,#190716,#190717,#190718,#190719,#190720,#190721,#190722,
#190723,#190724,#190725,#190726,#190727,#190728,#190729,#190730,#190731,
#190732,#190733,#190734,#190735,#190736,#190737,#190738,#190739,#190740,
#190741,#190742,#190743,#190744,#190745,#190746,#190747,#190748,#190749,
#190750,#190751),.UNSPECIFIED.,.F.,.F.,(4,3,3,3,3,3,3,3,3,3,3,3,3,3,3,3,
3,4),(0.,2.58457451676215E-5,4.25394446194861E-5,6.46659869686614E-5,7.5729258143249E-5,
8.12608937305428E-5,8.26438026273662E-5,8.67925293178366E-5,0.000116015624427751,
0.000130188793976755,0.000151886926306214,0.000161963651211277,0.000162735992470944,
0.000173585058635673,0.000212487880461416,0.00025523817351186,0.000301397761145538,
0.000347170117271364),.UNSPECIFIED.);
#4593=B_SPLINE_CURVE_WITH_KNOTS('',3,(#190753,#190754,#190755,#190756,#190757,
#190758,#190759,#190760,#190761,#190762,#190763,#190764,#190765,#190766,
#190767,#190768,#190769,#190770,#190771,#190772,#190773,#190774,#190775,
#190776,#190777,#190778,#190779,#190780,#190781,#190782,#190783,#190784,
#190785,#190786,#190787,#190788,#190789,#190790,#190791,#190792,#190793,
#190794,#190795,#190796,#190797,#190798),.UNSPECIFIED.,.F.,.F.,(4,3,3,3,
3,3,3,3,3,3,3,3,3,3,3,4),(0.,2.5721816201431E-5,4.2156832256571E-5,6.45873314615971E-5,
7.58025810641102E-5,8.14102058653667E-5,8.28121120656809E-5,8.70178306666232E-5,
0.000116081955658063,0.000130526745999935,0.000162394111022062,0.000174035661333246,
0.000213138396959622,0.000256116935436423,0.000302406662859842,0.00034807132266648),
 .UNSPECIFIED.);
#4594=B_SPLINE_CURVE_WITH_KNOTS('',3,(#190799,#190800,#190801,#190802,#190803,
#190804,#190805,#190806,#190807,#190808,#190809,#190810,#190811,#190812,
#190813,#190814,#190815,#190816,#190817,#190818,#190819,#190820,#190821,
#190822,#190823,#190824,#190825,#190826,#190827,#190828,#190829,#190830,
#190831,#190832,#190833,#190834,#190835,#190836,#190837,#190838,#190839,
#190840,#190841,#190842,#190843,#190844,#190845,#190846,#190847,#190848,
#190849,#190850),.UNSPECIFIED.,.F.,.F.,(4,3,3,3,3,3,3,3,3,3,3,3,3,3,3,3,
3,4),(0.,4.29652152174073E-5,8.44519107557636E-5,0.000123669830868272,0.000159788877362364,
0.000170558847912617,0.000181218775907158,0.000181960046452397,0.000214460062643918,
0.00024475572619964,0.00025583827186894,0.000258503253867575,0.000261084955178753,
0.000289370476646583,0.000301101325502008,0.000321109510663635,0.000331113603244449,
0.000341117695825263),.UNSPECIFIED.);
#4595=B_SPLINE_CURVE_WITH_KNOTS('',3,(#190852,#190853,#190854,#190855,#190856,
#190857,#190858,#190859,#190860,#190861,#190862,#190863,#190864,#190865,
#190866,#190867,#190868,#190869,#190870,#190871,#190872,#190873,#190874,
#190875,#190876,#190877,#190878,#190879,#190880,#190881,#190882,#190883,
#190884,#190885,#190886,#190887,#190888,#190889,#190890,#190891,#190892,
#190893,#190894,#190895,#190896,#190897,#190898,#190899,#190900,#190901,
#190902,#190903),.UNSPECIFIED.,.F.,.F.,(4,3,3,3,3,3,3,3,3,3,3,3,3,3,3,3,
3,4),(0.,4.30706237853522E-5,8.47417087667565E-5,0.000124159989201577,0.000160467076284533,
0.000170998382116685,0.000182414994733785,0.000213747977645861,0.000242415955903341,
0.000256497573175037,0.000259169422895611,0.000261757777312416,0.000289965130402767,
0.000301877270772903,0.000321937017503146,0.000326951954185707,0.000334474359209548,
0.00034199676423339),.UNSPECIFIED.);
#4596=B_SPLINE_CURVE_WITH_KNOTS('',3,(#190904,#190905,#190906,#190907,#190908,
#190909,#190910,#190911,#190912,#190913,#190914,#190915,#190916,#190917,
#190918,#190919,#190920,#190921,#190922,#190923,#190924,#190925,#190926,
#190927,#190928,#190929,#190930,#190931,#190932,#190933,#190934,#190935,
#190936,#190937,#190938,#190939,#190940,#190941,#190942,#190943,#190944,
#190945,#190946,#190947,#190948,#190949,#190950,#190951,#190952,#190953,
#190954,#190955),.UNSPECIFIED.,.F.,.F.,(4,3,3,3,3,3,3,3,3,3,3,3,3,3,3,3,
3,4),(0.,2.58457451685608E-5,4.25394446196307E-5,6.46659869687341E-5,7.57292581432858E-5,
8.12608937305616E-5,8.26438026273806E-5,8.67925293178375E-5,0.00011601562442651,
0.000130188793976756,0.000151886926306216,0.000161963651211271,0.000162735992470945,
0.000173585058635675,0.000212487880459305,0.00025523817350915,0.000301397761144963,
0.000347170117271364),.UNSPECIFIED.);
#4597=B_SPLINE_CURVE_WITH_KNOTS('',3,(#190957,#190958,#190959,#190960,#190961,
#190962,#190963,#190964,#190965,#190966,#190967,#190968,#190969,#190970,
#190971,#190972,#190973,#190974,#190975,#190976,#190977,#190978,#190979,
#190980,#190981,#190982,#190983,#190984,#190985,#190986,#190987,#190988,
#190989,#190990,#190991,#190992,#190993,#190994,#190995,#190996,#190997,
#190998,#190999,#191000,#191001,#191002),.UNSPECIFIED.,.F.,.F.,(4,3,3,3,
3,3,3,3,3,3,3,3,3,3,3,4),(0.,2.57218161988706E-5,4.21568322567235E-5,6.45873314616673E-5,
7.58025810641392E-5,8.14102058653752E-5,8.28121120656842E-5,8.70178306666111E-5,
0.00011608195565852,0.000130526745999917,0.000162394111022032,0.000174035661333222,
0.00021313839695844,0.000256116935434141,0.00030240666285643,0.000348071322666455),
 .UNSPECIFIED.);
#4598=B_SPLINE_CURVE_WITH_KNOTS('',3,(#191003,#191004,#191005,#191006,#191007,
#191008,#191009,#191010,#191011,#191012,#191013,#191014,#191015,#191016,
#191017,#191018,#191019,#191020,#191021,#191022,#191023,#191024,#191025,
#191026,#191027,#191028,#191029,#191030,#191031,#191032,#191033,#191034,
#191035,#191036,#191037,#191038,#191039,#191040,#191041,#191042,#191043,
#191044,#191045,#191046,#191047,#191048,#191049,#191050,#191051,#191052,
#191053,#191054),.UNSPECIFIED.,.F.,.F.,(4,3,3,3,3,3,3,3,3,3,3,3,3,3,3,3,
3,4),(0.,4.29652152136145E-5,8.44519107492294E-5,0.000123669830859522,0.000159788877351505,
0.000170558847912633,0.000181218775907172,0.000181960046452411,0.000214460062643391,
0.000244755726198025,0.000255838271868944,0.000258503253867578,0.000261084955178756,
0.000289370476648214,0.000301101325502005,0.000321109510663629,0.000331113603244442,
0.000341117695825254),.UNSPECIFIED.);
#4599=B_SPLINE_CURVE_WITH_KNOTS('',3,(#191056,#191057,#191058,#191059,#191060,
#191061,#191062,#191063,#191064,#191065,#191066,#191067,#191068,#191069,
#191070,#191071,#191072,#191073,#191074,#191075,#191076,#191077,#191078,
#191079,#191080,#191081,#191082,#191083,#191084,#191085,#191086,#191087,
#191088,#191089,#191090,#191091,#191092,#191093,#191094,#191095,#191096,
#191097,#191098,#191099,#191100,#191101,#191102,#191103,#191104,#191105,
#191106,#191107),.UNSPECIFIED.,.F.,.F.,(4,3,3,3,3,3,3,3,3,3,3,3,3,3,3,3,
3,4),(0.,4.3070623786896E-5,8.47417087695961E-5,0.000124159989205574,0.000160467076289785,
0.000170998382116694,0.00018241499473378,0.000213747977645867,0.000242415955902538,
0.000256497573175039,0.000259169422895613,0.000261757777312418,0.000289965130402436,
0.000301877270772901,0.000321937017503143,0.000326951954185703,0.000334474359209544,
0.000341996764233384),.UNSPECIFIED.);
#4600=B_SPLINE_CURVE_WITH_KNOTS('',3,(#191108,#191109,#191110,#191111,#191112,
#191113,#191114,#191115,#191116,#191117,#191118,#191119,#191120,#191121,
#191122,#191123,#191124,#191125,#191126,#191127,#191128,#191129,#191130,
#191131,#191132,#191133,#191134,#191135,#191136,#191137,#191138,#191139,
#191140,#191141,#191142,#191143,#191144,#191145,#191146,#191147,#191148,
#191149,#191150,#191151,#191152,#191153,#191154,#191155,#191156,#191157,
#191158,#191159),.UNSPECIFIED.,.F.,.F.,(4,3,3,3,3,3,3,3,3,3,3,3,3,3,3,3,
3,4),(0.,2.58457451667925E-5,4.25394446195448E-5,6.46659869686894E-5,7.57292581432617E-5,
8.12608937305479E-5,8.26438026273694E-5,8.6792529317834E-5,0.000116015624426846,
0.000130188793976751,0.00015188692630621,0.000161963651211258,0.000162735992470939,
0.000173585058635668,0.000212487880462275,0.000255238173515101,0.000301397761154326,
0.000347170117271365),.UNSPECIFIED.);
#4601=B_SPLINE_CURVE_WITH_KNOTS('',3,(#191161,#191162,#191163,#191164,#191165,
#191166,#191167,#191168,#191169,#191170,#191171,#191172,#191173,#191174,
#191175,#191176,#191177,#191178,#191179,#191180,#191181,#191182,#191183,
#191184,#191185,#191186,#191187,#191188,#191189,#191190,#191191,#191192,
#191193,#191194,#191195,#191196,#191197,#191198,#191199,#191200,#191201,
#191202,#191203,#191204,#191205,#191206),.UNSPECIFIED.,.F.,.F.,(4,3,3,3,
3,3,3,3,3,3,3,3,3,3,3,4),(0.,2.57218161986573E-5,4.21568322566464E-5,6.45873314616308E-5,
7.5802581064123E-5,8.14102058653691E-5,8.28121120656806E-5,8.70178306666152E-5,
0.00011608195565807,0.000130526745999923,0.000162394111022048,0.00017403566133323,
0.000213138396960761,0.000256116935438828,0.000302406662863967,0.000348071322666457),
 .UNSPECIFIED.);
#4602=B_SPLINE_CURVE_WITH_KNOTS('',3,(#191207,#191208,#191209,#191210,#191211,
#191212,#191213,#191214,#191215,#191216,#191217,#191218,#191219,#191220,
#191221,#191222,#191223,#191224,#191225,#191226,#191227,#191228,#191229,
#191230,#191231,#191232,#191233,#191234,#191235,#191236,#191237,#191238,
#191239,#191240,#191241,#191242,#191243,#191244,#191245,#191246,#191247,
#191248,#191249,#191250,#191251,#191252,#191253,#191254,#191255,#191256,
#191257,#191258),.UNSPECIFIED.,.F.,.F.,(4,3,3,3,3,3,3,3,3,3,3,3,3,3,3,3,
3,4),(0.,4.296521522581E-5,8.44519107689155E-5,0.000123669830883573,0.000159788877378198,
0.000170558847912618,0.000181218775907158,0.000181960046452403,0.000214460062644037,
0.000244755726199692,0.000255838271868937,0.000258503253867572,0.00026108495517875,
0.000289370476646679,0.000301101325502003,0.00032110951066363,0.000331113603244443,
0.000341117695825257),.UNSPECIFIED.);
#4603=B_SPLINE_CURVE_WITH_KNOTS('',3,(#191260,#191261,#191262,#191263,#191264,
#191265,#191266,#191267,#191268,#191269,#191270,#191271,#191272,#191273,
#191274,#191275,#191276,#191277,#191278,#191279,#191280,#191281,#191282,
#191283,#191284,#191285,#191286,#191287,#191288,#191289,#191290,#191291,
#191292,#191293,#191294,#191295,#191296,#191297,#191298,#191299,#191300,
#191301,#191302,#191303,#191304,#191305,#191306,#191307,#191308,#191309,
#191310,#191311),.UNSPECIFIED.,.F.,.F.,(4,3,3,3,3,3,3,3,3,3,3,3,3,3,3,3,
3,4),(2.23960286815172E-17,4.30706237876585E-5,8.47417087709534E-5,0.000124159989207585,
0.00016046707629245,0.000170998382116699,0.000182414994733791,0.000213747977645874,
0.000242415955903611,0.000256497573175049,0.000259169422895623,0.000261757777312428,
0.000289965130403366,0.000301877270772914,0.000321937017503157,0.000326951954185718,
0.000334474359209559,0.0003419967642334),.UNSPECIFIED.);
#4604=B_SPLINE_CURVE_WITH_KNOTS('',3,(#191312,#191313,#191314,#191315,#191316,
#191317,#191318,#191319,#191320,#191321,#191322,#191323,#191324,#191325,
#191326,#191327,#191328,#191329,#191330,#191331,#191332,#191333,#191334,
#191335,#191336,#191337,#191338,#191339,#191340,#191341,#191342,#191343,
#191344,#191345,#191346,#191347,#191348,#191349,#191350,#191351,#191352,
#191353,#191354,#191355,#191356,#191357,#191358,#191359,#191360,#191361,
#191362,#191363),.UNSPECIFIED.,.F.,.F.,(4,3,3,3,3,3,3,3,3,3,3,3,3,3,3,3,
3,4),(0.,2.58457451680856E-5,4.25394446195527E-5,6.46659869687014E-5,7.57292581432757E-5,
8.12608937305629E-5,8.26438026273847E-5,8.67925293178501E-5,0.000116015624427437,
0.000130188793976775,0.000151886926306238,0.000161963651211304,0.000162735992470969,
0.0001735850586357,0.000212487880459721,0.000255238173510426,0.000301397761147914,
0.000347170117271371),.UNSPECIFIED.);
#4605=B_SPLINE_CURVE_WITH_KNOTS('',3,(#191365,#191366,#191367,#191368,#191369,
#191370,#191371,#191372,#191373,#191374,#191375,#191376,#191377,#191378,
#191379,#191380,#191381,#191382,#191383,#191384,#191385,#191386,#191387,
#191388,#191389,#191390,#191391,#191392,#191393,#191394,#191395,#191396,
#191397,#191398,#191399,#191400,#191401,#191402,#191403,#191404,#191405,
#191406,#191407,#191408,#191409,#191410),.UNSPECIFIED.,.F.,.F.,(4,3,3,3,
3,3,3,3,3,3,3,3,3,3,3,4),(3.46944695195361E-18,2.57218162016344E-5,4.21568322567852E-5,
6.45873314617071E-5,7.58025810641681E-5,8.14102058653986E-5,8.28121120657062E-5,
8.70178306666291E-5,0.000116081955658797,0.000130526745999942,0.000162394111022068,
0.000174035661333255,0.000213138396959518,0.000256116935436304,0.000302406662860053,
0.000348071322666477),.UNSPECIFIED.);
#4606=B_SPLINE_CURVE_WITH_KNOTS('',3,(#191411,#191412,#191413,#191414,#191415,
#191416,#191417,#191418,#191419,#191420,#191421,#191422,#191423,#191424,
#191425,#191426,#191427,#191428,#191429,#191430,#191431,#191432,#191433,
#191434,#191435,#191436,#191437,#191438,#191439,#191440,#191441,#191442,
#191443,#191444,#191445,#191446,#191447,#191448,#191449,#191450,#191451,
#191452,#191453,#191454,#191455,#191456,#191457,#191458,#191459,#191460,
#191461,#191462),.UNSPECIFIED.,.F.,.F.,(4,3,3,3,3,3,3,3,3,3,3,3,3,3,3,3,
3,4),(0.,4.2965215215576E-5,8.44519107527791E-5,0.000123669830864603,0.00015978887735827,
0.000170558847912638,0.000181218775907178,0.000181960046452423,0.00021446006264388,
0.000244755726199131,0.000255838271868956,0.000258503253867591,0.000261084955178768,
0.000289370476647343,0.000301101325502021,0.000321109510663647,0.00033111360324446,
0.000341117695825273),.UNSPECIFIED.);
#4607=B_SPLINE_CURVE_WITH_KNOTS('',3,(#191464,#191465,#191466,#191467,#191468,
#191469,#191470,#191471,#191472,#191473,#191474,#191475,#191476,#191477,
#191478,#191479,#191480,#191481,#191482,#191483,#191484,#191485,#191486,
#191487,#191488,#191489,#191490,#191491,#191492,#191493,#191494,#191495,
#191496,#191497,#191498,#191499,#191500,#191501,#191502,#191503,#191504,
#191505,#191506,#191507,#191508,#191509,#191510,#191511,#191512,#191513,
#191514,#191515),.UNSPECIFIED.,.F.,.F.,(4,3,3,3,3,3,3,3,3,3,3,3,3,3,3,3,
3,4),(0.,4.30706237881386E-5,8.47417087717555E-5,0.000124159989208601,0.000160467076293699,
0.000170998382116686,0.000182414994733776,0.000213747977645861,0.000242415955903616,
0.000256497573175037,0.00025916942289561,0.000261757777312415,0.000289965130402526,
0.000301877270772901,0.000321937017503144,0.000326951954185705,0.000334474359209546,
0.000341996764233387),.UNSPECIFIED.);
#4608=B_SPLINE_CURVE_WITH_KNOTS('',3,(#191516,#191517,#191518,#191519,#191520,
#191521,#191522,#191523,#191524,#191525,#191526,#191527,#191528,#191529,
#191530,#191531,#191532,#191533,#191534,#191535,#191536,#191537,#191538,
#191539,#191540,#191541,#191542,#191543,#191544,#191545,#191546,#191547,
#191548,#191549,#191550,#191551,#191552,#191553,#191554,#191555,#191556,
#191557,#191558,#191559,#191560,#191561,#191562,#191563,#191564,#191565,
#191566,#191567),.UNSPECIFIED.,.F.,.F.,(4,3,3,3,3,3,3,3,3,3,3,3,3,3,3,3,
3,4),(0.,2.584574516724E-5,4.25394446196669E-5,6.46659869687501E-5,7.57292581432917E-5,
8.12608937305625E-5,8.26438026273802E-5,8.67925293178333E-5,0.000116015624427194,
0.00013018879397675,0.000151886926306208,0.000161963651211274,0.000162735992470937,
0.000173585058635667,0.000212487880460265,0.000255238173511465,0.000301397761149537,
0.00034717011727135),.UNSPECIFIED.);
#4609=B_SPLINE_CURVE_WITH_KNOTS('',3,(#191569,#191570,#191571,#191572,#191573,
#191574,#191575,#191576,#191577,#191578,#191579,#191580,#191581,#191582,
#191583,#191584,#191585,#191586,#191587,#191588,#191589,#191590,#191591,
#191592,#191593,#191594,#191595,#191596,#191597,#191598,#191599,#191600,
#191601,#191602,#191603,#191604,#191605,#191606,#191607,#191608,#191609,
#191610,#191611,#191612,#191613,#191614),.UNSPECIFIED.,.F.,.F.,(4,3,3,3,
3,3,3,3,3,3,3,3,3,3,3,4),(1.73472347597681E-18,2.57218162000535E-5,4.21568322566752E-5,
6.45873314616487E-5,7.58025810641355E-5,8.14102058653789E-5,8.28121120656897E-5,
8.70178306666222E-5,0.000116081955659069,0.000130526745999932,0.000162394111022052,
0.000174035661333243,0.000213138396958092,0.000256116935433535,0.000302406662855884,
0.000348071322666481),.UNSPECIFIED.);
#4610=B_SPLINE_CURVE_WITH_KNOTS('',3,(#191615,#191616,#191617,#191618,#191619,
#191620,#191621,#191622,#191623,#191624,#191625,#191626,#191627,#191628,
#191629,#191630,#191631,#191632,#191633,#191634,#191635,#191636,#191637,
#191638,#191639,#191640,#191641,#191642,#191643,#191644,#191645,#191646,
#191647,#191648,#191649,#191650,#191651,#191652,#191653,#191654,#191655,
#191656,#191657,#191658,#191659,#191660,#191661,#191662,#191663,#191664,
#191665,#191666),.UNSPECIFIED.,.F.,.F.,(4,3,3,3,3,3,3,3,3,3,3,3,3,3,3,3,
3,4),(0.,4.29652152124446E-5,8.44519107478593E-5,0.000123669830858857,0.000159788877352283,
0.000170558847912616,0.000181218775907156,0.000181960046452394,0.000214460062644285,
0.000244755726200151,0.000255838271868935,0.00025850325386757,0.000261084955178748,
0.000289370476646895,0.000301101325502001,0.000321109510663628,0.000331113603244441,
0.000341117695825255),.UNSPECIFIED.);
#4611=B_SPLINE_CURVE_WITH_KNOTS('',3,(#191668,#191669,#191670,#191671,#191672,
#191673,#191674,#191675,#191676,#191677,#191678,#191679,#191680,#191681,
#191682,#191683,#191684,#191685,#191686,#191687,#191688,#191689,#191690,
#191691,#191692,#191693,#191694,#191695,#191696,#191697,#191698,#191699,
#191700,#191701,#191702,#191703,#191704,#191705,#191706,#191707,#191708,
#191709,#191710,#191711,#191712,#191713,#191714,#191715,#191716,#191717,
#191718,#191719),.UNSPECIFIED.,.F.,.F.,(4,3,3,3,3,3,3,3,3,3,3,3,3,3,3,3,
3,4),(0.,4.3070623786735E-5,8.47417087692355E-5,0.000124159989205176,0.00016046707628918,
0.000170998382116699,0.000182414994733791,0.000213747977645873,0.000242415955904601,
0.000256497573175047,0.00025916942289562,0.000261757777312426,0.000289965130402128,
0.000301877270772907,0.000321937017503148,0.000326951954185708,0.000334474359209548,
0.000341996764233388),.UNSPECIFIED.);
#4612=B_SPLINE_CURVE_WITH_KNOTS('',3,(#191720,#191721,#191722,#191723,#191724,
#191725,#191726,#191727,#191728,#191729,#191730,#191731,#191732,#191733,
#191734,#191735,#191736,#191737,#191738,#191739,#191740,#191741,#191742,
#191743,#191744,#191745,#191746,#191747,#191748,#191749,#191750,#191751,
#191752,#191753,#191754,#191755,#191756,#191757,#191758,#191759,#191760,
#191761,#191762,#191763,#191764,#191765,#191766,#191767,#191768,#191769,
#191770,#191771),.UNSPECIFIED.,.F.,.F.,(4,3,3,3,3,3,3,3,3,3,3,3,3,3,3,3,
3,4),(0.,2.58457451678823E-5,4.25394446195921E-5,6.46659869687165E-5,7.57292581432787E-5,
8.12608937305598E-5,8.26438026273801E-5,8.67925293178409E-5,0.00011601562442684,
0.000130188793976761,0.000151886926306222,0.000161963651211289,0.000162735992470952,
0.000173585058635682,0.000212487880460706,0.00025523817351073,0.000301397761144501,
0.000347170117271364),.UNSPECIFIED.);
#4613=B_SPLINE_CURVE_WITH_KNOTS('',3,(#191773,#191774,#191775,#191776,#191777,
#191778,#191779,#191780,#191781,#191782,#191783,#191784,#191785,#191786,
#191787,#191788,#191789,#191790,#191791,#191792,#191793,#191794,#191795,
#191796,#191797,#191798,#191799,#191800,#191801,#191802,#191803,#191804,
#191805,#191806,#191807,#191808,#191809,#191810,#191811,#191812,#191813,
#191814,#191815,#191816,#191817,#191818),.UNSPECIFIED.,.F.,.F.,(4,3,3,3,
3,3,3,3,3,3,3,3,3,3,3,4),(1.73472347597681E-18,2.57218161989433E-5,4.21568322567811E-5,
6.45873314617046E-5,7.58025810641663E-5,8.14102058653971E-5,8.28121120657048E-5,
8.7017830666628E-5,0.000116081955658619,0.000130526745999941,0.000162394111022059,
0.000174035661333254,0.000213138396960531,0.00025611693543839,0.000302406662863409,
0.000348071322666518),.UNSPECIFIED.);
#4614=B_SPLINE_CURVE_WITH_KNOTS('',3,(#191819,#191820,#191821,#191822,#191823,
#191824,#191825,#191826,#191827,#191828,#191829,#191830,#191831,#191832,
#191833,#191834,#191835,#191836,#191837,#191838,#191839,#191840,#191841,
#191842,#191843,#191844,#191845,#191846,#191847,#191848,#191849,#191850,
#191851,#191852,#191853,#191854,#191855,#191856,#191857,#191858,#191859,
#191860,#191861,#191862,#191863,#191864,#191865,#191866,#191867,#191868,
#191869,#191870),.UNSPECIFIED.,.F.,.F.,(4,3,3,3,3,3,3,3,3,3,3,3,3,3,3,3,
3,4),(0.,4.29652152204607E-5,8.44519107603203E-5,0.000123669830873161,0.000159788877366737,
0.000170558847912626,0.000181218775907165,0.000181960046452412,0.000214460062644189,
0.000244755726200295,0.000255838271868945,0.00025850325386758,0.000261084955178758,
0.000289370476646845,0.000301101325502011,0.000321109510663638,0.000331113603244451,
0.000341117695825265),.UNSPECIFIED.);
#4615=B_SPLINE_CURVE_WITH_KNOTS('',3,(#191872,#191873,#191874,#191875,#191876,
#191877,#191878,#191879,#191880,#191881,#191882,#191883,#191884,#191885,
#191886,#191887,#191888,#191889,#191890,#191891,#191892,#191893,#191894,
#191895,#191896,#191897,#191898,#191899,#191900,#191901,#191902,#191903,
#191904,#191905,#191906,#191907,#191908,#191909,#191910,#191911,#191912,
#191913,#191914,#191915,#191916,#191917,#191918,#191919,#191920,#191921,
#191922,#191923),.UNSPECIFIED.,.F.,.F.,(4,3,3,3,3,3,3,3,3,3,3,3,3,3,3,3,
3,4),(0.,4.3070623786749E-5,8.4741708769304E-5,0.000124159989205248,0.000160467076289362,
0.000170998382116684,0.000182414994733762,0.000213747977645858,0.00024241595590281,
0.000256497573175033,0.000259169422895606,0.000261757777312412,0.000289965130403439,
0.000301877270772897,0.000321937017503139,0.0003269519541857,0.000334474359209541,
0.000341996764233382),.UNSPECIFIED.);
#4616=B_SPLINE_CURVE_WITH_KNOTS('',3,(#191924,#191925,#191926,#191927,#191928,
#191929,#191930,#191931,#191932,#191933,#191934,#191935,#191936,#191937,
#191938,#191939,#191940,#191941,#191942,#191943,#191944,#191945,#191946,
#191947,#191948,#191949,#191950,#191951,#191952,#191953,#191954,#191955,
#191956,#191957,#191958,#191959,#191960,#191961,#191962,#191963,#191964,
#191965,#191966,#191967,#191968,#191969,#191970,#191971,#191972,#191973,
#191974,#191975),.UNSPECIFIED.,.F.,.F.,(4,3,3,3,3,3,3,3,3,3,3,3,3,3,3,3,
3,4),(0.,2.58457451687104E-5,4.25394446195245E-5,6.46659869686809E-5,7.57292581432591E-5,
8.12608937305483E-5,8.26438026273705E-5,8.67925293178374E-5,0.000116015624427198,
0.000130188793976756,0.000151886926306215,0.000161963651211279,0.000162735992470945,
0.000173585058635675,0.000212487880460741,0.000255238173511971,0.000301397761149513,
0.00034717011727135),.UNSPECIFIED.);
#4617=B_SPLINE_CURVE_WITH_KNOTS('',3,(#191977,#191978,#191979,#191980,#191981,
#191982,#191983,#191984,#191985,#191986,#191987,#191988,#191989,#191990,
#191991,#191992,#191993,#191994,#191995,#191996,#191997,#191998,#191999,
#192000,#192001,#192002,#192003,#192004,#192005,#192006,#192007,#192008,
#192009,#192010,#192011,#192012,#192013,#192014,#192015,#192016,#192017,
#192018,#192019,#192020,#192021,#192022),.UNSPECIFIED.,.F.,.F.,(4,3,3,3,
3,3,3,3,3,3,3,3,3,3,3,4),(5.48877349820787E-19,2.57218161989097E-5,4.2156832256823E-5,
6.45873314617228E-5,7.58025810641727E-5,8.14102058653976E-5,8.28121120657039E-5,
8.70178306666226E-5,0.000116081955657846,0.000130526745999934,0.000162394111022054,
0.000174035661333245,0.000213138396957884,0.000256116935433115,0.000302406662855211,
0.000348071322666501),.UNSPECIFIED.);
#4618=B_SPLINE_CURVE_WITH_KNOTS('',3,(#192023,#192024,#192025,#192026,#192027,
#192028,#192029,#192030,#192031,#192032,#192033,#192034,#192035,#192036,
#192037,#192038,#192039,#192040,#192041,#192042,#192043,#192044,#192045,
#192046,#192047,#192048,#192049,#192050,#192051,#192052,#192053,#192054,
#192055,#192056,#192057,#192058,#192059,#192060,#192061,#192062,#192063,
#192064,#192065,#192066,#192067,#192068,#192069,#192070,#192071,#192072,
#192073,#192074),.UNSPECIFIED.,.F.,.F.,(4,3,3,3,3,3,3,3,3,3,3,3,3,3,3,3,
3,4),(0.,4.29652152190797E-5,8.44519107582085E-5,0.000123669830870829,0.000159788877364511,
0.000170558847912623,0.000181218775907163,0.000181960046452403,0.000214460062643601,
0.000244755726198573,0.000255838271868941,0.000258503253867576,0.000261084955178753,
0.000289370476648259,0.000301101325502006,0.000321109510663632,0.000331113603244445,
0.000341117695825259),.UNSPECIFIED.);
#4619=B_SPLINE_CURVE_WITH_KNOTS('',3,(#192076,#192077,#192078,#192079,#192080,
#192081,#192082,#192083,#192084,#192085,#192086,#192087,#192088,#192089,
#192090,#192091,#192092,#192093,#192094,#192095,#192096,#192097,#192098,
#192099,#192100,#192101,#192102,#192103,#192104,#192105,#192106,#192107,
#192108,#192109,#192110,#192111,#192112,#192113,#192114,#192115,#192116,
#192117,#192118,#192119,#192120,#192121,#192122,#192123,#192124,#192125,
#192126,#192127),.UNSPECIFIED.,.F.,.F.,(4,3,3,3,3,3,3,3,3,3,3,3,3,3,3,3,
3,4),(9.85133562538035E-18,4.30706237855933E-5,8.47417087672294E-5,0.000124159989202406,
0.000160467076285688,0.000170998382116695,0.000182414994733793,0.000213747977645867,
0.000242415955902541,0.000256497573175038,0.000259169422895611,0.000261757777312417,
0.00028996513040345,0.000301877270772899,0.00032193701750314,0.0003269519541857,
0.00033447435920954,0.000341996764233381),.UNSPECIFIED.);
#4620=B_SPLINE_CURVE_WITH_KNOTS('',3,(#192128,#192129,#192130,#192131,#192132,
#192133,#192134,#192135,#192136,#192137,#192138,#192139,#192140,#192141,
#192142,#192143,#192144,#192145,#192146,#192147,#192148,#192149,#192150,
#192151,#192152,#192153,#192154,#192155,#192156,#192157,#192158,#192159,
#192160,#192161,#192162,#192163,#192164,#192165,#192166,#192167,#192168,
#192169,#192170,#192171,#192172,#192173,#192174,#192175,#192176,#192177,
#192178,#192179),.UNSPECIFIED.,.F.,.F.,(4,3,3,3,3,3,3,3,3,3,3,3,3,3,3,3,
3,4),(0.,2.58457451673525E-5,4.25394446195986E-5,6.46659869687198E-5,7.57292581432803E-5,
8.12608937305606E-5,8.26438026273807E-5,8.67925293178409E-5,0.000116015624426975,
0.000130188793976761,0.000151886926306222,0.000161963651211268,0.000162735992470952,
0.000173585058635682,0.000212487880460807,0.00025523817351178,0.000301397761147946,
0.000347170117271376),.UNSPECIFIED.);
#4621=B_SPLINE_CURVE_WITH_KNOTS('',3,(#192181,#192182,#192183,#192184,#192185,
#192186,#192187,#192188,#192189,#192190,#192191,#192192,#192193,#192194,
#192195,#192196,#192197,#192198,#192199,#192200,#192201,#192202,#192203,
#192204,#192205,#192206,#192207,#192208,#192209,#192210,#192211,#192212,
#192213,#192214,#192215,#192216,#192217,#192218,#192219,#192220,#192221,
#192222,#192223,#192224,#192225,#192226),.UNSPECIFIED.,.F.,.F.,(4,3,3,3,
3,3,3,3,3,3,3,3,3,3,3,4),(8.67361737988403E-19,2.57218161984597E-5,4.21568322567013E-5,
6.45873314616616E-5,7.58025810641418E-5,8.14102058653818E-5,8.28121120656919E-5,
8.70178306666219E-5,0.000116081955658696,0.000130526745999929,0.000162394111022049,
0.000174035661333235,0.00021313839696006,0.000256116935437399,0.00030240666286165,
0.000348071322666489),.UNSPECIFIED.);
#4622=B_SPLINE_CURVE_WITH_KNOTS('',3,(#192227,#192228,#192229,#192230,#192231,
#192232,#192233,#192234,#192235,#192236,#192237,#192238,#192239,#192240,
#192241,#192242,#192243,#192244,#192245,#192246,#192247,#192248,#192249,
#192250,#192251,#192252,#192253,#192254,#192255,#192256,#192257,#192258,
#192259,#192260,#192261,#192262,#192263,#192264,#192265,#192266,#192267,
#192268,#192269,#192270,#192271,#192272,#192273,#192274,#192275,#192276,
#192277,#192278),.UNSPECIFIED.,.F.,.F.,(4,3,3,3,3,3,3,3,3,3,3,3,3,3,3,3,
3,4),(0.,4.29652152191222E-5,8.44519107581807E-5,0.000123669830870584,0.000159788877363929,
0.000170558847912617,0.000181218775907157,0.0001819600464524,0.000214460062643968,
0.000244755726199534,0.000255838271868939,0.000258503253867574,0.000261084955178751,
0.000289370476646808,0.000301101325502006,0.000321109510663633,0.000331113603244447,
0.00034111769582526),.UNSPECIFIED.);
#4623=B_SPLINE_CURVE_WITH_KNOTS('',3,(#192280,#192281,#192282,#192283,#192284,
#192285,#192286,#192287,#192288,#192289,#192290,#192291,#192292,#192293,
#192294,#192295,#192296,#192297,#192298,#192299,#192300,#192301,#192302,
#192303,#192304,#192305,#192306,#192307,#192308,#192309,#192310,#192311,
#192312,#192313,#192314,#192315,#192316,#192317,#192318,#192319,#192320,
#192321,#192322,#192323,#192324,#192325,#192326,#192327,#192328,#192329,
#192330,#192331),.UNSPECIFIED.,.F.,.F.,(4,3,3,3,3,3,3,3,3,3,3,3,3,3,3,3,
3,4),(0.,4.30706237878556E-5,8.47417087713877E-5,0.000124159989208393,0.000160467076293688,
0.000170998382116697,0.000182414994733767,0.000213747977645869,0.000242415955903676,
0.000256497573175041,0.000259169422895614,0.000261757777312419,0.000289965130402761,
0.000301877270772902,0.000321937017503143,0.000326951954185703,0.000334474359209544,
0.000341996764233384),.UNSPECIFIED.);
#4624=B_SPLINE_CURVE_WITH_KNOTS('',3,(#192332,#192333,#192334,#192335,#192336,
#192337,#192338,#192339,#192340,#192341,#192342,#192343,#192344,#192345,
#192346,#192347,#192348,#192349,#192350,#192351,#192352,#192353,#192354,
#192355,#192356,#192357,#192358,#192359,#192360,#192361,#192362,#192363,
#192364,#192365,#192366,#192367,#192368,#192369,#192370,#192371,#192372,
#192373,#192374,#192375,#192376,#192377,#192378,#192379,#192380,#192381,
#192382,#192383),.UNSPECIFIED.,.F.,.F.,(4,3,3,3,3,3,3,3,3,3,3,3,3,3,3,3,
3,4),(0.,2.5845745168666E-5,4.25394446195824E-5,6.46659869687127E-5,7.57292581432779E-5,
8.12608937305605E-5,8.26438026273811E-5,8.6792529317843E-5,0.000116015624428386,
0.000130188793976765,0.000151886926306225,0.000161963651211285,0.000162735992470956,
0.000173585058635686,0.000212487880463336,0.00025523817351687,0.000301397761156083,
0.000347170117271363),.UNSPECIFIED.);
#4625=B_SPLINE_CURVE_WITH_KNOTS('',3,(#192385,#192386,#192387,#192388,#192389,
#192390,#192391,#192392,#192393,#192394,#192395,#192396,#192397,#192398,
#192399,#192400,#192401,#192402,#192403,#192404,#192405,#192406,#192407,
#192408,#192409,#192410,#192411,#192412,#192413,#192414,#192415,#192416,
#192417,#192418,#192419,#192420,#192421,#192422,#192423,#192424,#192425,
#192426,#192427,#192428,#192429,#192430),.UNSPECIFIED.,.F.,.F.,(4,3,3,3,
3,3,3,3,3,3,3,3,3,3,3,4),(0.,2.57218161995338E-5,4.21568322567715E-5,6.45873314616955E-5,
7.58025810641576E-5,8.14102058653886E-5,8.28121120656963E-5,8.70178306666196E-5,
0.000116081955657908,0.000130526745999929,0.000162394111022051,0.000174035661333239,
0.000213138396960905,0.000256116935439096,0.0003024066628643,0.000348071322666476),
 .UNSPECIFIED.);
#4626=B_SPLINE_CURVE_WITH_KNOTS('',3,(#192431,#192432,#192433,#192434,#192435,
#192436,#192437,#192438,#192439,#192440,#192441,#192442,#192443,#192444,
#192445,#192446,#192447,#192448,#192449,#192450,#192451,#192452,#192453,
#192454,#192455,#192456,#192457,#192458,#192459,#192460,#192461,#192462,
#192463,#192464,#192465,#192466,#192467,#192468,#192469,#192470,#192471,
#192472,#192473,#192474,#192475,#192476,#192477,#192478,#192479,#192480,
#192481,#192482),.UNSPECIFIED.,.F.,.F.,(4,3,3,3,3,3,3,3,3,3,3,3,3,3,3,3,
3,4),(0.,4.29652152168045E-5,8.44519107545815E-5,0.000123669830866463,0.000159788877359758,
0.000170558847912623,0.000181218775907163,0.000181960046452399,0.000214460062643643,
0.000244755726198916,0.000255838271868941,0.000258503253867576,0.000261084955178754,
0.000289370476647759,0.000301101325502006,0.000321109510663633,0.000331113603244446,
0.000341117695825259),.UNSPECIFIED.);
#4627=B_SPLINE_CURVE_WITH_KNOTS('',3,(#192484,#192485,#192486,#192487,#192488,
#192489,#192490,#192491,#192492,#192493,#192494,#192495,#192496,#192497,
#192498,#192499,#192500,#192501,#192502,#192503,#192504,#192505,#192506,
#192507,#192508,#192509,#192510,#192511,#192512,#192513,#192514,#192515,
#192516,#192517,#192518,#192519,#192520,#192521,#192522,#192523,#192524,
#192525,#192526,#192527,#192528,#192529,#192530,#192531,#192532,#192533,
#192534,#192535),.UNSPECIFIED.,.F.,.F.,(4,3,3,3,3,3,3,3,3,3,3,3,3,3,3,3,
3,4),(0.,4.30706237843463E-5,8.47417087647801E-5,0.000124159989198604,0.000160467076280188,
0.000170998382116709,0.000182414994733815,0.00021374797764588,0.00024241595590353,
0.000256497573175051,0.000259169422895624,0.000261757777312429,0.000289965130403544,
0.000301877270772911,0.000321937017503151,0.000326951954185712,0.000334474359209552,
0.000341996764233392),.UNSPECIFIED.);
#4628=B_SPLINE_CURVE_WITH_KNOTS('',3,(#192536,#192537,#192538,#192539,#192540,
#192541,#192542,#192543,#192544,#192545,#192546,#192547,#192548,#192549,
#192550,#192551,#192552,#192553,#192554,#192555,#192556,#192557,#192558,
#192559,#192560,#192561,#192562,#192563,#192564,#192565,#192566,#192567,
#192568,#192569,#192570,#192571,#192572,#192573,#192574,#192575,#192576,
#192577,#192578,#192579,#192580,#192581,#192582,#192583,#192584,#192585,
#192586,#192587),.UNSPECIFIED.,.F.,.F.,(4,3,3,3,3,3,3,3,3,3,3,3,3,3,3,3,
3,4),(0.,2.58457451680454E-5,4.25394446195865E-5,6.46659869687126E-5,7.57292581432756E-5,
8.12608937305571E-5,8.26438026273775E-5,8.67925293178386E-5,0.000116015624427228,
0.000130188793976758,0.000151886926306218,0.000161963651211266,0.000162735992470947,
0.000173585058635677,0.00021248788045917,0.000255238173507915,0.000301397761140769,
0.000347170117271374),.UNSPECIFIED.);
#4629=B_SPLINE_CURVE_WITH_KNOTS('',3,(#192589,#192590,#192591,#192592,#192593,
#192594,#192595,#192596,#192597,#192598,#192599,#192600,#192601,#192602,
#192603,#192604,#192605,#192606,#192607,#192608,#192609,#192610,#192611,
#192612,#192613,#192614,#192615,#192616,#192617,#192618,#192619,#192620,
#192621,#192622,#192623,#192624,#192625,#192626,#192627,#192628,#192629,
#192630,#192631,#192632,#192633,#192634),.UNSPECIFIED.,.F.,.F.,(4,3,3,3,
3,3,3,3,3,3,3,3,3,3,3,4),(0.,2.57218162011368E-5,4.21568322568854E-5,6.45873314617514E-5,
7.58025810641844E-5,8.14102058654009E-5,8.2812112065705E-5,8.70178306666174E-5,
0.000116081955658846,0.000130526745999926,0.000162394111022064,0.000174035661333235,
0.000213138396958756,0.000256116935434756,0.000302406662857426,0.000348071322666454),
 .UNSPECIFIED.);
#4630=B_SPLINE_CURVE_WITH_KNOTS('',3,(#192635,#192636,#192637,#192638,#192639,
#192640,#192641,#192642,#192643,#192644,#192645,#192646,#192647,#192648,
#192649,#192650,#192651,#192652,#192653,#192654,#192655,#192656,#192657,
#192658,#192659,#192660,#192661,#192662,#192663,#192664,#192665,#192666,
#192667,#192668,#192669,#192670,#192671,#192672,#192673,#192674,#192675,
#192676,#192677,#192678,#192679,#192680,#192681,#192682,#192683,#192684,
#192685,#192686),.UNSPECIFIED.,.F.,.F.,(4,3,3,3,3,3,3,3,3,3,3,3,3,3,3,3,
3,4),(0.,4.29652152214354E-5,8.44519107622748E-5,0.000123669830876302,0.00015978887737137,
0.000170558847912627,0.000181218775907166,0.000181960046452393,0.000214460062643908,
0.000244755726199127,0.000255838271868937,0.000258503253867572,0.000261084955178749,
0.000289370476646983,0.000301101325501999,0.000321109510663623,0.000331113603244436,
0.000341117695825248),.UNSPECIFIED.);
#4631=B_SPLINE_CURVE_WITH_KNOTS('',3,(#192688,#192689,#192690,#192691,#192692,
#192693,#192694,#192695,#192696,#192697,#192698,#192699,#192700,#192701,
#192702,#192703,#192704,#192705,#192706,#192707,#192708,#192709,#192710,
#192711,#192712,#192713,#192714,#192715,#192716,#192717,#192718,#192719,
#192720,#192721,#192722,#192723,#192724,#192725,#192726,#192727,#192728,
#192729,#192730,#192731,#192732,#192733,#192734,#192735,#192736,#192737,
#192738,#192739),.UNSPECIFIED.,.F.,.F.,(4,3,3,3,3,3,3,3,3,3,3,3,3,3,3,3,
3,4),(0.,4.30706237879649E-5,8.47417087713518E-5,0.000124159989207974,0.000160467076292721,
0.000170998382116688,0.000182414994733775,0.000213747977645863,0.000242415955903171,
0.000256497573175039,0.000259169422895612,0.000261757777312418,0.000289965130403515,
0.000301877270772904,0.000321937017503147,0.000326951954185707,0.000334474359209549,
0.00034199676423339),.UNSPECIFIED.);
#4632=B_SPLINE_CURVE_WITH_KNOTS('',3,(#192740,#192741,#192742,#192743,#192744,
#192745,#192746,#192747,#192748,#192749,#192750,#192751,#192752,#192753,
#192754,#192755,#192756,#192757,#192758,#192759,#192760,#192761,#192762,
#192763,#192764,#192765,#192766,#192767,#192768,#192769,#192770,#192771,
#192772,#192773,#192774,#192775,#192776,#192777,#192778,#192779,#192780,
#192781,#192782,#192783,#192784,#192785,#192786,#192787,#192788,#192789,
#192790,#192791),.UNSPECIFIED.,.F.,.F.,(4,3,3,3,3,3,3,3,3,3,3,3,3,3,3,3,
3,4),(0.,2.58457451674872E-5,4.25394446196628E-5,6.46659869687521E-5,7.57292581432967E-5,
8.12608937305691E-5,8.26438026273871E-5,8.67925293178414E-5,0.000116015624427357,
0.000130188793976762,0.000151886926306222,0.000161963651211285,0.000162735992470953,
0.000173585058635683,0.000212487880460278,0.00025523817350991,0.000301397761143294,
0.000347170117271361),.UNSPECIFIED.);
#4633=B_SPLINE_CURVE_WITH_KNOTS('',3,(#192793,#192794,#192795,#192796,#192797,
#192798,#192799,#192800,#192801,#192802,#192803,#192804,#192805,#192806,
#192807,#192808,#192809,#192810,#192811,#192812,#192813,#192814,#192815,
#192816,#192817,#192818,#192819,#192820,#192821,#192822,#192823,#192824,
#192825,#192826,#192827,#192828,#192829,#192830,#192831,#192832,#192833,
#192834,#192835,#192836,#192837,#192838),.UNSPECIFIED.,.F.,.F.,(4,3,3,3,
3,3,3,3,3,3,3,3,3,3,3,4),(3.46944695195361E-18,2.57218162008425E-5,4.21568322567336E-5,
6.45873314616739E-5,7.58025810641441E-5,8.14102058653791E-5,8.28121120656879E-5,
8.70178306666142E-5,0.000116081955659379,0.00013052674599992,0.000162394111022033,
0.000174035661333225,0.000213138396959368,0.000256116935436057,0.000302406662859663,
0.00034807132266646),.UNSPECIFIED.);
#4634=B_SPLINE_CURVE_WITH_KNOTS('',3,(#192839,#192840,#192841,#192842,#192843,
#192844,#192845,#192846,#192847,#192848,#192849,#192850,#192851,#192852,
#192853,#192854,#192855,#192856,#192857,#192858,#192859,#192860,#192861,
#192862,#192863,#192864,#192865,#192866,#192867,#192868,#192869,#192870,
#192871,#192872,#192873,#192874,#192875,#192876,#192877,#192878,#192879,
#192880,#192881,#192882,#192883,#192884,#192885,#192886,#192887,#192888,
#192889,#192890),.UNSPECIFIED.,.F.,.F.,(4,3,3,3,3,3,3,3,3,3,3,3,3,3,3,3,
3,4),(0.,4.29652152146269E-5,8.44519107510616E-5,0.000123669830862063,0.000159788877354834,
0.000170558847912627,0.000181218775907166,0.000181960046452403,0.000214460062643365,
0.0002447557261976,0.000255838271868941,0.000258503253867576,0.000261084955178753,
0.000289370476647798,0.000301101325502004,0.00032110951066363,0.000331113603244442,
0.000341117695825255),.UNSPECIFIED.);
#4635=B_SPLINE_CURVE_WITH_KNOTS('',3,(#192892,#192893,#192894,#192895,#192896,
#192897,#192898,#192899,#192900,#192901,#192902,#192903,#192904,#192905,
#192906,#192907,#192908,#192909,#192910,#192911,#192912,#192913,#192914,
#192915,#192916,#192917,#192918,#192919,#192920,#192921,#192922,#192923,
#192924,#192925,#192926,#192927,#192928,#192929,#192930,#192931,#192932,
#192933,#192934,#192935,#192936,#192937,#192938,#192939,#192940,#192941,
#192942,#192943),.UNSPECIFIED.,.F.,.F.,(4,3,3,3,3,3,3,3,3,3,3,3,3,3,3,3,
3,4),(0.,4.30706237882749E-5,8.47417087721192E-5,0.000124159989209344,0.000160467076294915,
0.000170998382116705,0.000182414994733787,0.000213747977645879,0.00024241595590288,
0.000256497573175053,0.000259169422895626,0.000261757777312432,0.000289965130402957,
0.000301877270772916,0.000321937017503158,0.000326951954185719,0.00033447435920956,
0.0003419967642334),.UNSPECIFIED.);
#4636=B_SPLINE_CURVE_WITH_KNOTS('',3,(#192944,#192945,#192946,#192947,#192948,
#192949,#192950,#192951,#192952,#192953,#192954,#192955,#192956,#192957,
#192958,#192959,#192960,#192961,#192962,#192963,#192964,#192965,#192966,
#192967,#192968,#192969,#192970,#192971,#192972,#192973,#192974,#192975,
#192976,#192977,#192978,#192979,#192980,#192981,#192982,#192983,#192984,
#192985,#192986,#192987,#192988,#192989,#192990,#192991,#192992,#192993,
#192994,#192995),.UNSPECIFIED.,.F.,.F.,(4,3,3,3,3,3,3,3,3,3,3,3,3,3,3,3,
3,4),(0.,2.58457451677947E-5,4.25394446196165E-5,6.46659869687299E-5,7.57292581432866E-5,
8.12608937305649E-5,8.26438026273845E-5,8.67925293178432E-5,0.000116015624427386,
0.000130188793976765,0.000151886926306226,0.000161963651211264,0.000162735992470956,
0.000173585058635686,0.00021248788045667,0.000255238173502178,0.000301397761129961,
0.000347170117271371),.UNSPECIFIED.);
#4637=B_SPLINE_CURVE_WITH_KNOTS('',3,(#192997,#192998,#192999,#193000,#193001,
#193002,#193003,#193004,#193005,#193006,#193007,#193008,#193009,#193010,
#193011,#193012,#193013,#193014,#193015,#193016,#193017,#193018,#193019,
#193020,#193021,#193022,#193023,#193024,#193025,#193026,#193027,#193028,
#193029,#193030,#193031,#193032,#193033,#193034,#193035,#193036,#193037,
#193038,#193039,#193040,#193041,#193042),.UNSPECIFIED.,.F.,.F.,(4,3,3,3,
3,3,3,3,3,3,3,3,3,3,3,4),(0.,2.57218161985032E-5,4.21568322569506E-5,6.45873314617842E-5,
7.5802581064201E-5,8.14102058654094E-5,8.28121120657115E-5,8.70178306666178E-5,
0.00011608195565788,0.000130526745999927,0.000162394111022043,0.000174035661333236,
0.000213138396958693,0.000256116935434544,0.000302406662856772,0.000348071322666484),
 .UNSPECIFIED.);
#4638=B_SPLINE_CURVE_WITH_KNOTS('',3,(#193043,#193044,#193045,#193046,#193047,
#193048,#193049,#193050,#193051,#193052,#193053,#193054,#193055,#193056,
#193057,#193058,#193059,#193060,#193061,#193062,#193063,#193064,#193065,
#193066,#193067,#193068,#193069,#193070,#193071,#193072,#193073,#193074,
#193075,#193076,#193077,#193078,#193079,#193080,#193081,#193082,#193083,
#193084,#193085,#193086,#193087,#193088,#193089,#193090,#193091,#193092,
#193093,#193094),.UNSPECIFIED.,.F.,.F.,(4,3,3,3,3,3,3,3,3,3,3,3,3,3,3,3,
3,4),(0.,4.29652152129906E-5,8.44519107478209E-5,0.000123669830856864,0.000159788877347059,
0.000170558847912636,0.000181218775907175,0.000181960046452432,0.000214460062643819,
0.000244755726198886,0.000255838271868951,0.000258503253867586,0.000261084955178763,
0.000289370476647964,0.000301101325502015,0.00032110951066364,0.000331113603244453,
0.000341117695825266),.UNSPECIFIED.);
#4639=B_SPLINE_CURVE_WITH_KNOTS('',3,(#193096,#193097,#193098,#193099,#193100,
#193101,#193102,#193103,#193104,#193105,#193106,#193107,#193108,#193109,
#193110,#193111,#193112,#193113,#193114,#193115,#193116,#193117,#193118,
#193119,#193120,#193121,#193122,#193123,#193124,#193125,#193126,#193127,
#193128,#193129,#193130,#193131,#193132,#193133,#193134,#193135,#193136,
#193137,#193138,#193139,#193140,#193141,#193142,#193143,#193144,#193145,
#193146,#193147),.UNSPECIFIED.,.F.,.F.,(4,3,3,3,3,3,3,3,3,3,3,3,3,3,3,3,
3,4),(0.,4.3070623787665E-5,8.47417087708582E-5,0.000124159989207229,0.000160467076291828,
0.000170998382116699,0.000182414994733755,0.000213747977645872,0.000242415955902611,
0.000256497573175046,0.000259169422895619,0.000261757777312424,0.000289965130403524,
0.000301877270772909,0.000321937017503151,0.000326951954185711,0.000334474359209552,
0.000341996764233393),.UNSPECIFIED.);
#4640=B_SPLINE_CURVE_WITH_KNOTS('',3,(#193148,#193149,#193150,#193151,#193152,
#193153,#193154,#193155,#193156,#193157,#193158,#193159,#193160,#193161,
#193162,#193163,#193164,#193165,#193166,#193167,#193168,#193169,#193170,
#193171,#193172,#193173,#193174,#193175,#193176,#193177,#193178,#193179,
#193180,#193181,#193182,#193183,#193184,#193185,#193186,#193187,#193188,
#193189,#193190,#193191,#193192,#193193,#193194,#193195,#193196,#193197,
#193198,#193199),.UNSPECIFIED.,.F.,.F.,(4,3,3,3,3,3,3,3,3,3,3,3,3,3,3,3,
3,4),(0.,2.58457451692331E-5,4.25394446195874E-5,6.46659869687102E-5,7.57292581432715E-5,
8.12608937305522E-5,8.26438026273724E-5,8.67925293178329E-5,0.000116015624428751,
0.000130188793976749,0.000151886926306208,0.000161963651211278,0.000162735992470937,
0.000173585058635666,0.000212487880459203,0.000255238173507225,0.000301397761137999,
0.000347170117271348),.UNSPECIFIED.);
#4641=B_SPLINE_CURVE_WITH_KNOTS('',3,(#193201,#193202,#193203,#193204,#193205,
#193206,#193207,#193208,#193209,#193210,#193211,#193212,#193213,#193214,
#193215,#193216,#193217,#193218,#193219,#193220,#193221,#193222,#193223,
#193224,#193225,#193226,#193227,#193228,#193229,#193230,#193231,#193232,
#193233,#193234,#193235,#193236,#193237,#193238,#193239,#193240,#193241,
#193242,#193243,#193244,#193245,#193246),.UNSPECIFIED.,.F.,.F.,(4,3,3,3,
3,3,3,3,3,3,3,3,3,3,3,4),(6.93889390390723E-18,2.57218162003168E-5,4.2156832256597E-5,
6.45873314616125E-5,7.58025810641203E-5,8.14102058653742E-5,8.28121120656877E-5,
8.70178306666281E-5,0.000116081955659664,0.000130526745999939,0.000162394111022071,
0.000174035661333249,0.000213138396962072,0.000256116935441266,0.000302406662867136,
0.000348071322666479),.UNSPECIFIED.);
#4642=B_SPLINE_CURVE_WITH_KNOTS('',3,(#193247,#193248,#193249,#193250,#193251,
#193252,#193253,#193254,#193255,#193256,#193257,#193258,#193259,#193260,
#193261,#193262,#193263,#193264,#193265,#193266,#193267,#193268,#193269,
#193270,#193271,#193272,#193273,#193274,#193275,#193276,#193277,#193278,
#193279,#193280,#193281,#193282,#193283,#193284,#193285,#193286,#193287,
#193288,#193289,#193290,#193291,#193292,#193293,#193294,#193295,#193296,
#193297,#193298),.UNSPECIFIED.,.F.,.F.,(4,3,3,3,3,3,3,3,3,3,3,3,3,3,3,3,
3,4),(0.,4.29652152181114E-5,8.44519107563061E-5,0.000123669830867864,0.000159788877360231,
0.00017055884791263,0.000181218775907169,0.000181960046452423,0.000214460062643701,
0.000244755726198761,0.000255838271868939,0.000258503253867574,0.000261084955178751,
0.000289370476648725,0.000301101325502,0.000321109510663624,0.000331113603244436,
0.000341117695825248),.UNSPECIFIED.);
#4643=B_SPLINE_CURVE_WITH_KNOTS('',3,(#193300,#193301,#193302,#193303,#193304,
#193305,#193306,#193307,#193308,#193309,#193310,#193311,#193312,#193313,
#193314,#193315,#193316,#193317,#193318,#193319,#193320,#193321,#193322,
#193323,#193324,#193325,#193326,#193327,#193328,#193329,#193330,#193331,
#193332,#193333,#193334,#193335,#193336,#193337,#193338,#193339,#193340,
#193341,#193342,#193343,#193344,#193345,#193346,#193347,#193348,#193349,
#193350,#193351),.UNSPECIFIED.,.F.,.F.,(4,3,3,3,3,3,3,3,3,3,3,3,3,3,3,3,
3,4),(0.,4.30706237873436E-5,8.47417087703543E-5,0.000124159989206768,0.000160467076291368,
0.000170998382116691,0.000182414994733778,0.000213747977645865,0.000242415955903022,
0.000256497573175039,0.000259169422895612,0.000261757777312417,0.000289965130402893,
0.000301877270772902,0.000321937017503144,0.000326951954185705,0.000334474359209545,
0.000341996764233386),.UNSPECIFIED.);
#4644=B_SPLINE_CURVE_WITH_KNOTS('',3,(#193352,#193353,#193354,#193355,#193356,
#193357,#193358,#193359,#193360,#193361,#193362,#193363,#193364,#193365,
#193366,#193367,#193368,#193369,#193370,#193371,#193372,#193373,#193374,
#193375,#193376,#193377,#193378,#193379,#193380,#193381,#193382,#193383,
#193384,#193385,#193386,#193387,#193388,#193389,#193390,#193391,#193392,
#193393,#193394,#193395,#193396,#193397,#193398,#193399,#193400,#193401,
#193402,#193403),.UNSPECIFIED.,.F.,.F.,(4,3,3,3,3,3,3,3,3,3,3,3,3,3,3,3,
3,4),(0.,2.58457451679608E-5,4.25394446195563E-5,6.46659869686995E-5,7.57292581432711E-5,
8.12608937305569E-5,8.26438026273783E-5,8.67925293178427E-5,0.000116015624427097,
0.000130188793976764,0.000151886926306225,0.000161963651211274,0.000162735992470955,
0.000173585058635685,0.000212487880461448,0.000255238173513823,0.000301397761153107,
0.000347170117271366),.UNSPECIFIED.);
#4645=B_SPLINE_CURVE_WITH_KNOTS('',3,(#193405,#193406,#193407,#193408,#193409,
#193410,#193411,#193412,#193413,#193414,#193415,#193416,#193417,#193418,
#193419,#193420,#193421,#193422,#193423,#193424,#193425,#193426,#193427,
#193428,#193429,#193430,#193431,#193432,#193433,#193434,#193435,#193436,
#193437,#193438,#193439,#193440,#193441,#193442,#193443,#193444,#193445,
#193446,#193447,#193448,#193449,#193450),.UNSPECIFIED.,.F.,.F.,(4,3,3,3,
3,3,3,3,3,3,3,3,3,3,3,4),(0.,2.57218162026608E-5,4.21568322568483E-5,6.45873314617269E-5,
7.58025810641662E-5,8.14102058653858E-5,8.28121120656908E-5,8.70178306666055E-5,
0.00011608195565896,0.000130526745999908,0.000162394111022025,0.000174035661333211,
0.000213138396955903,0.000256116935429113,0.000302406662848748,0.000348071322666448),
 .UNSPECIFIED.);
#4646=B_SPLINE_CURVE_WITH_KNOTS('',3,(#193451,#193452,#193453,#193454,#193455,
#193456,#193457,#193458,#193459,#193460,#193461,#193462,#193463,#193464,
#193465,#193466,#193467,#193468,#193469,#193470,#193471,#193472,#193473,
#193474,#193475,#193476,#193477,#193478,#193479,#193480,#193481,#193482,
#193483,#193484,#193485,#193486,#193487,#193488,#193489,#193490,#193491,
#193492,#193493,#193494,#193495,#193496,#193497,#193498,#193499,#193500,
#193501,#193502),.UNSPECIFIED.,.F.,.F.,(4,3,3,3,3,3,3,3,3,3,3,3,3,3,3,3,
3,4),(0.,4.29652152145236E-5,8.44519107509453E-5,0.000123669830862064,0.00015978887735497,
0.000170558847912636,0.000181218775907175,0.00018196004645242,0.000214460062643987,
0.000244755726199668,0.000255838271868951,0.000258503253867586,0.000261084955178763,
0.000289370476647399,0.000301101325502015,0.000321109510663641,0.000331113603244453,
0.000341117695825266),.UNSPECIFIED.);
#4647=B_SPLINE_CURVE_WITH_KNOTS('',3,(#193504,#193505,#193506,#193507,#193508,
#193509,#193510,#193511,#193512,#193513,#193514,#193515,#193516,#193517,
#193518,#193519,#193520,#193521,#193522,#193523,#193524,#193525,#193526,
#193527,#193528,#193529,#193530,#193531,#193532,#193533,#193534,#193535,
#193536,#193537,#193538,#193539,#193540,#193541,#193542,#193543,#193544,
#193545,#193546,#193547,#193548,#193549,#193550,#193551,#193552,#193553,
#193554,#193555),.UNSPECIFIED.,.F.,.F.,(4,3,3,3,3,3,3,3,3,3,3,3,3,3,3,3,
3,4),(0.,4.30706237867132E-5,8.47417087692055E-5,0.000124159989205097,0.000160467076289105,
0.000170998382116699,0.00018241499473378,0.000213747977645872,0.000242415955902537,
0.000256497573175045,0.000259169422895618,0.000261757777312424,0.000289965130403846,
0.000301877270772907,0.000321937017503149,0.000326951954185709,0.00033447435920955,
0.000341996764233391),.UNSPECIFIED.);
#4648=B_SPLINE_CURVE_WITH_KNOTS('',3,(#193556,#193557,#193558,#193559,#193560,
#193561,#193562,#193563,#193564,#193565,#193566,#193567,#193568,#193569,
#193570,#193571,#193572,#193573,#193574,#193575,#193576,#193577,#193578,
#193579,#193580,#193581,#193582,#193583,#193584,#193585,#193586,#193587,
#193588,#193589,#193590,#193591,#193592,#193593,#193594,#193595,#193596,
#193597,#193598,#193599,#193600,#193601,#193602,#193603,#193604,#193605,
#193606,#193607),.UNSPECIFIED.,.F.,.F.,(4,3,3,3,3,3,3,3,3,3,3,3,3,3,3,3,
3,4),(0.,2.58457451670712E-5,4.25394446195834E-5,6.46659869687109E-5,7.57292581432746E-5,
8.12608937305565E-5,8.26438026273769E-5,8.67925293178383E-5,0.000116015624426661,
0.000130188793976757,0.000151886926306217,0.000161963651211276,0.000162735992470947,
0.000173585058635677,0.000212487880459323,0.000255238173507097,0.00030139776113686,
0.000347170117271366),.UNSPECIFIED.);
#4649=B_SPLINE_CURVE_WITH_KNOTS('',3,(#193609,#193610,#193611,#193612,#193613,
#193614,#193615,#193616,#193617,#193618,#193619,#193620,#193621,#193622,
#193623,#193624,#193625,#193626,#193627,#193628,#193629,#193630,#193631,
#193632,#193633,#193634,#193635,#193636,#193637,#193638,#193639,#193640,
#193641,#193642,#193643,#193644,#193645,#193646,#193647,#193648,#193649,
#193650,#193651,#193652,#193653,#193654),.UNSPECIFIED.,.F.,.F.,(4,3,3,3,
3,3,3,3,3,3,3,3,3,3,3,4),(0.,2.57218161984597E-5,4.21568322568931E-5,6.45873314617548E-5,
7.58025810641856E-5,8.1410205865401E-5,8.28121120657048E-5,8.70178306666164E-5,
0.000116081955658237,0.000130526745999925,0.000162394111022039,0.000174035661333233,
0.0002131383969588,0.000256116935434844,0.000302406662857505,0.000348071322666477),
 .UNSPECIFIED.);
#4650=B_SPLINE_CURVE_WITH_KNOTS('',3,(#193655,#193656,#193657,#193658,#193659,
#193660,#193661,#193662,#193663,#193664,#193665,#193666,#193667,#193668,
#193669,#193670,#193671,#193672,#193673,#193674,#193675,#193676,#193677,
#193678,#193679,#193680,#193681,#193682,#193683,#193684,#193685,#193686,
#193687,#193688,#193689,#193690,#193691,#193692,#193693,#193694,#193695,
#193696,#193697,#193698,#193699,#193700,#193701,#193702,#193703,#193704,
#193705,#193706),.UNSPECIFIED.,.F.,.F.,(4,3,3,3,3,3,3,3,3,3,3,3,3,3,3,3,
3,4),(0.,4.29652152191473E-5,8.44519107585247E-5,0.000123669830871658,0.000159788877366025,
0.000170558847912618,0.000181218775907159,0.0001819600464524,0.000214460062643458,
0.000244755726197822,0.000255838271868943,0.000258503253867578,0.000261084955178756,
0.000289370476647256,0.000301101325502011,0.000321109510663639,0.000331113603244453,
0.000341117695825267),.UNSPECIFIED.);
#4651=B_SPLINE_CURVE_WITH_KNOTS('',3,(#193708,#193709,#193710,#193711,#193712,
#193713,#193714,#193715,#193716,#193717,#193718,#193719,#193720,#193721,
#193722,#193723,#193724,#193725,#193726,#193727,#193728,#193729,#193730,
#193731,#193732,#193733,#193734,#193735,#193736,#193737,#193738,#193739,
#193740,#193741,#193742,#193743,#193744,#193745,#193746,#193747,#193748,
#193749,#193750,#193751,#193752,#193753,#193754,#193755,#193756,#193757,
#193758,#193759),.UNSPECIFIED.,.F.,.F.,(4,3,3,3,3,3,3,3,3,3,3,3,3,3,3,3,
3,4),(0.,4.30706237879909E-5,8.47417087713626E-5,0.000124159989208026,0.000160467076292825,
0.000170998382116693,0.000182414994733774,0.000213747977645869,0.000242415955903556,
0.000256497573175044,0.000259169422895617,0.000261757777312423,0.000289965130402278,
0.000301877270772909,0.000321937017503151,0.000326951954185712,0.000334474359209553,
0.000341996764233394),.UNSPECIFIED.);
#4652=B_SPLINE_CURVE_WITH_KNOTS('',3,(#193760,#193761,#193762,#193763,#193764,
#193765,#193766,#193767,#193768,#193769,#193770,#193771,#193772,#193773,
#193774,#193775,#193776,#193777,#193778,#193779,#193780,#193781,#193782,
#193783,#193784,#193785,#193786,#193787,#193788,#193789,#193790,#193791,
#193792,#193793,#193794,#193795,#193796,#193797,#193798,#193799,#193800,
#193801,#193802,#193803,#193804,#193805,#193806,#193807,#193808,#193809,
#193810,#193811),.UNSPECIFIED.,.F.,.F.,(4,3,3,3,3,3,3,3,3,3,3,3,3,3,3,3,
3,4),(0.,2.58457451684838E-5,4.25394446196393E-5,6.46659869687357E-5,7.5729258143284E-5,
8.12608937305581E-5,8.26438026273766E-5,8.67925293178322E-5,0.000116015624428102,
0.000130188793976748,0.000151886926306206,0.000161963651211262,0.000162735992470935,
0.000173585058635664,0.000212487880461562,0.000255238173513034,0.000301397761149555,
0.000347170117271345),.UNSPECIFIED.);
#4653=B_SPLINE_CURVE_WITH_KNOTS('',3,(#193813,#193814,#193815,#193816,#193817,
#193818,#193819,#193820,#193821,#193822,#193823,#193824,#193825,#193826,
#193827,#193828,#193829,#193830,#193831,#193832,#193833,#193834,#193835,
#193836,#193837,#193838,#193839,#193840,#193841,#193842,#193843,#193844,
#193845,#193846,#193847,#193848,#193849,#193850,#193851,#193852,#193853,
#193854,#193855,#193856,#193857,#193858),.UNSPECIFIED.,.F.,.F.,(4,3,3,3,
3,3,3,3,3,3,3,3,3,3,3,4),(0.,2.57218162004422E-5,4.21568322566571E-5,6.45873314616386E-5,
7.58025810641293E-5,8.14102058653747E-5,8.2812112065686E-5,8.701783066662E-5,
0.000116081955658433,0.00013052674599993,0.000162394111022039,0.00017403566133324,
0.000213138396960911,0.00025611693543884,0.00030240666286298,0.000348071322666468),
 .UNSPECIFIED.);
#4654=B_SPLINE_CURVE_WITH_KNOTS('',3,(#193859,#193860,#193861,#193862,#193863,
#193864,#193865,#193866,#193867,#193868,#193869,#193870,#193871,#193872,
#193873,#193874,#193875,#193876,#193877,#193878,#193879,#193880,#193881,
#193882,#193883,#193884,#193885,#193886,#193887,#193888,#193889,#193890,
#193891,#193892,#193893,#193894,#193895,#193896,#193897,#193898,#193899,
#193900,#193901,#193902,#193903,#193904,#193905,#193906,#193907,#193908,
#193909,#193910),.UNSPECIFIED.,.F.,.F.,(4,3,3,3,3,3,3,3,3,3,3,3,3,3,3,3,
3,4),(0.,4.2965215219619E-5,8.44519107588242E-5,0.000123669830871205,0.000159788877364292,
0.000170558847912618,0.000181218775907158,0.000181960046452387,0.000214460062643356,
0.000244755726198647,0.000255838271868941,0.000258503253867576,0.000261084955178754,
0.000289370476647944,0.000301101325502009,0.000321109510663637,0.00033111360324445,
0.000341117695825264),.UNSPECIFIED.);
#4655=B_SPLINE_CURVE_WITH_KNOTS('',3,(#193912,#193913,#193914,#193915,#193916,
#193917,#193918,#193919,#193920,#193921,#193922,#193923,#193924,#193925,
#193926,#193927,#193928,#193929,#193930,#193931,#193932,#193933,#193934,
#193935,#193936,#193937,#193938,#193939,#193940,#193941,#193942,#193943,
#193944,#193945,#193946,#193947,#193948,#193949,#193950,#193951,#193952,
#193953,#193954,#193955,#193956,#193957,#193958,#193959,#193960,#193961,
#193962,#193963),.UNSPECIFIED.,.F.,.F.,(4,3,3,3,3,3,3,3,3,3,3,3,3,3,3,3,
3,4),(0.,4.30706237860952E-5,8.47417087682543E-5,0.000124159989203998,0.000160467076288037,
0.000170998382116714,0.000182414994733819,0.000213747977645884,0.000242415955903088,
0.000256497573175054,0.000259169422895627,0.000261757777312432,0.00028996513040302,
0.000301877270772912,0.000321937017503153,0.000326951954185713,0.000334474359209553,
0.000341996764233393),.UNSPECIFIED.);
#4656=B_SPLINE_CURVE_WITH_KNOTS('',3,(#193964,#193965,#193966,#193967,#193968,
#193969,#193970,#193971,#193972,#193973,#193974,#193975,#193976,#193977,
#193978,#193979,#193980,#193981,#193982,#193983,#193984,#193985,#193986,
#193987,#193988,#193989,#193990,#193991,#193992,#193993,#193994,#193995,
#193996,#193997,#193998,#193999,#194000,#194001,#194002,#194003,#194004,
#194005,#194006,#194007,#194008,#194009,#194010,#194011,#194012,#194013,
#194014,#194015),.UNSPECIFIED.,.F.,.F.,(4,3,3,3,3,3,3,3,3,3,3,3,3,3,3,3,
3,4),(0.,2.58457451687623E-5,4.25394446196227E-5,6.46659869687286E-5,7.57292581432816E-5,
8.12608937305581E-5,8.26438026273772E-5,8.67925293178346E-5,0.000116015624427777,
0.000130188793976752,0.000151886926306211,0.000161963651211265,0.00016273599247094,
0.000173585058635669,0.000212487880462122,0.000255238173513666,0.000301397761149318,
0.000347170117271352),.UNSPECIFIED.);
#4657=B_SPLINE_CURVE_WITH_KNOTS('',3,(#194017,#194018,#194019,#194020,#194021,
#194022,#194023,#194024,#194025,#194026,#194027,#194028,#194029,#194030,
#194031,#194032,#194033,#194034,#194035,#194036,#194037,#194038,#194039,
#194040,#194041,#194042,#194043,#194044,#194045,#194046,#194047,#194048,
#194049,#194050,#194051,#194052,#194053,#194054,#194055,#194056,#194057,
#194058,#194059,#194060,#194061,#194062),.UNSPECIFIED.,.F.,.F.,(4,3,3,3,
3,3,3,3,3,3,3,3,3,3,3,4),(0.,2.57218161985908E-5,4.21568322566518E-5,6.45873314616328E-5,
7.58025810641234E-5,8.14102058653686E-5,8.28121120656799E-5,8.70178306666139E-5,
0.000116081955657255,0.000130526745999921,0.000162394111022039,0.000174035661333228,
0.000213138396959342,0.000256116935435933,0.000302406662859232,0.000348071322666485),
 .UNSPECIFIED.);
#4658=B_SPLINE_CURVE_WITH_KNOTS('',3,(#194063,#194064,#194065,#194066,#194067,
#194068,#194069,#194070,#194071,#194072,#194073,#194074,#194075,#194076,
#194077,#194078,#194079,#194080,#194081,#194082,#194083,#194084,#194085,
#194086,#194087,#194088,#194089,#194090,#194091,#194092,#194093,#194094,
#194095,#194096,#194097,#194098,#194099,#194100,#194101,#194102,#194103,
#194104,#194105,#194106,#194107,#194108,#194109,#194110,#194111,#194112,
#194113,#194114),.UNSPECIFIED.,.F.,.F.,(4,3,3,3,3,3,3,3,3,3,3,3,3,3,3,3,
3,4),(0.,4.29652152172666E-5,8.44519107551468E-5,0.000123669830866818,0.000159788877359668,
0.000170558847912628,0.000181218775907168,0.000181960046452396,0.000214460062643525,
0.000244755726198588,0.000255838271868947,0.000258503253867582,0.00026108495517876,
0.000289370476648551,0.000301101325502014,0.000321109510663641,0.000331113603244454,
0.000341117695825267),.UNSPECIFIED.);
#4659=B_SPLINE_CURVE_WITH_KNOTS('',3,(#194116,#194117,#194118,#194119,#194120,
#194121,#194122,#194123,#194124,#194125,#194126,#194127,#194128,#194129,
#194130,#194131,#194132,#194133,#194134,#194135,#194136,#194137,#194138,
#194139,#194140,#194141,#194142,#194143,#194144,#194145,#194146,#194147,
#194148,#194149,#194150,#194151,#194152,#194153,#194154,#194155,#194156,
#194157,#194158,#194159,#194160,#194161,#194162,#194163,#194164,#194165,
#194166,#194167),.UNSPECIFIED.,.F.,.F.,(4,3,3,3,3,3,3,3,3,3,3,3,3,3,3,3,
3,4),(3.46944695195361E-18,4.30706237857577E-5,8.4741708767591E-5,0.000124159989202823,
0.000160467076286219,0.000170998382116696,0.000182414994733758,0.00021374797764587,
0.000242415955904134,0.000256497573175044,0.000259169422895617,0.000261757777312423,
0.000289965130402185,0.000301877270772907,0.00032193701750315,0.00032695195418571,
0.000334474359209551,0.000341996764233392),.UNSPECIFIED.);
#4660=B_SPLINE_CURVE_WITH_KNOTS('',3,(#194168,#194169,#194170,#194171,#194172,
#194173,#194174,#194175,#194176,#194177,#194178,#194179,#194180,#194181,
#194182,#194183,#194184,#194185,#194186,#194187,#194188,#194189,#194190,
#194191,#194192,#194193,#194194,#194195,#194196,#194197,#194198,#194199,
#194200,#194201,#194202,#194203,#194204,#194205,#194206,#194207,#194208,
#194209,#194210,#194211,#194212,#194213,#194214,#194215,#194216,#194217,
#194218,#194219),.UNSPECIFIED.,.F.,.F.,(4,3,3,3,3,3,3,3,3,3,3,3,3,3,3,3,
3,4),(0.,2.58457451699863E-5,4.25394446196659E-5,6.46659869687493E-5,7.5729258143291E-5,
8.12608937305619E-5,8.26438026273796E-5,8.67925293178327E-5,0.000116015624429004,
0.000130188793976749,0.000151886926306207,0.000161963651211244,0.000162735992470936,
0.000173585058635665,0.000212487880462874,0.000255238173516106,0.000301397761155294,
0.00034717011727135),.UNSPECIFIED.);
#4661=B_SPLINE_CURVE_WITH_KNOTS('',3,(#194221,#194222,#194223,#194224,#194225,
#194226,#194227,#194228,#194229,#194230,#194231,#194232,#194233,#194234,
#194235,#194236,#194237,#194238,#194239,#194240,#194241,#194242,#194243,
#194244,#194245,#194246,#194247,#194248,#194249,#194250,#194251,#194252,
#194253,#194254,#194255,#194256,#194257,#194258,#194259,#194260,#194261,
#194262,#194263,#194264,#194265,#194266),.UNSPECIFIED.,.F.,.F.,(4,3,3,3,
3,3,3,3,3,3,3,3,3,3,3,4),(3.46944695195361E-18,2.57218161988661E-5,4.21568322568949E-5,
6.45873314617574E-5,7.58025810641886E-5,8.14102058654043E-5,8.28121120657082E-5,
8.70178306666199E-5,0.000116081955658138,0.000130526745999928,0.000162394111022053,
0.000174035661333236,0.000213138396955745,0.000256116935428962,0.000302406662849146,
0.000348071322666463),.UNSPECIFIED.);
#4662=B_SPLINE_CURVE_WITH_KNOTS('',3,(#194267,#194268,#194269,#194270,#194271,
#194272,#194273,#194274,#194275,#194276,#194277,#194278,#194279,#194280,
#194281,#194282,#194283,#194284,#194285,#194286,#194287,#194288,#194289,
#194290,#194291,#194292,#194293,#194294,#194295,#194296,#194297,#194298,
#194299,#194300,#194301,#194302,#194303,#194304,#194305,#194306,#194307,
#194308,#194309,#194310,#194311,#194312,#194313,#194314,#194315,#194316,
#194317,#194318),.UNSPECIFIED.,.F.,.F.,(4,3,3,3,3,3,3,3,3,3,3,3,3,3,3,3,
3,4),(0.,4.29652152205376E-5,8.44519107610295E-5,0.000123669830875294,0.000159788877370972,
0.000170558847912616,0.000181218775907156,0.000181960046452398,0.000214460062644455,
0.000244755726200831,0.000255838271868934,0.000258503253867569,0.000261084955178747,
0.000289370476647454,0.000301101325502,0.000321109510663626,0.000331113603244439,
0.000341117695825252),.UNSPECIFIED.);
#4663=B_SPLINE_CURVE_WITH_KNOTS('',3,(#194320,#194321,#194322,#194323,#194324,
#194325,#194326,#194327,#194328,#194329,#194330,#194331,#194332,#194333,
#194334,#194335,#194336,#194337,#194338,#194339,#194340,#194341,#194342,
#194343,#194344,#194345,#194346,#194347,#194348,#194349,#194350,#194351,
#194352,#194353,#194354,#194355,#194356,#194357,#194358,#194359,#194360,
#194361,#194362,#194363,#194364,#194365,#194366,#194367,#194368,#194369,
#194370,#194371),.UNSPECIFIED.,.F.,.F.,(4,3,3,3,3,3,3,3,3,3,3,3,3,3,3,3,
3,4),(0.,4.30706237863112E-5,8.47417087684205E-5,0.000124159989203888,0.000160467076287372,
0.000170998382116698,0.00018241499473378,0.000213747977645872,0.000242415955903452,
0.000256497573175046,0.000259169422895619,0.000261757777312424,0.000289965130402983,
0.000301877270772909,0.000321937017503151,0.000326951954185711,0.000334474359209552,
0.000341996764233393),.UNSPECIFIED.);
#4664=B_SPLINE_CURVE_WITH_KNOTS('',3,(#194372,#194373,#194374,#194375,#194376,
#194377,#194378,#194379,#194380,#194381,#194382,#194383,#194384,#194385,
#194386,#194387,#194388,#194389,#194390,#194391,#194392,#194393,#194394,
#194395,#194396,#194397,#194398,#194399,#194400,#194401,#194402,#194403,
#194404,#194405,#194406,#194407,#194408,#194409,#194410,#194411,#194412,
#194413,#194414,#194415,#194416,#194417,#194418,#194419,#194420,#194421,
#194422,#194423),.UNSPECIFIED.,.F.,.F.,(4,3,3,3,3,3,3,3,3,3,3,3,3,3,3,3,
3,4),(3.46944695195361E-18,2.5845745168372E-5,4.25394446194478E-5,6.46659869686474E-5,
7.57292581432472E-5,8.12608937305471E-5,8.26438026273721E-5,8.6792529317847E-5,
0.000116015624428185,0.000130188793976769,0.00015188692630623,0.000161963651211288,
0.00016273599247096,0.000173585058635691,0.000212487880457827,0.000255238173505098,
0.000301397761135908,0.000347170117271362),.UNSPECIFIED.);
#4665=B_SPLINE_CURVE_WITH_KNOTS('',3,(#194425,#194426,#194427,#194428,#194429,
#194430,#194431,#194432,#194433,#194434,#194435,#194436,#194437,#194438,
#194439,#194440,#194441,#194442,#194443,#194444,#194445,#194446,#194447,
#194448,#194449,#194450,#194451,#194452,#194453,#194454,#194455,#194456,
#194457,#194458,#194459,#194460,#194461,#194462,#194463,#194464,#194465,
#194466,#194467,#194468,#194469,#194470),.UNSPECIFIED.,.F.,.F.,(4,3,3,3,
3,3,3,3,3,3,3,3,3,3,3,4),(3.46944695195361E-18,2.57218161998776E-5,4.21568322567625E-5,
6.45873314616899E-5,7.58025810641537E-5,8.14102058653855E-5,8.28121120656935E-5,
8.70178306666174E-5,0.000116081955658038,0.000130526745999924,0.000162394111022039,
0.000174035661333231,0.000213138396958318,0.000256116935433942,0.00030240666285635,
0.000348071322666463),.UNSPECIFIED.);
#4666=B_SPLINE_CURVE_WITH_KNOTS('',3,(#194471,#194472,#194473,#194474,#194475,
#194476,#194477,#194478,#194479,#194480,#194481,#194482,#194483,#194484,
#194485,#194486,#194487,#194488,#194489,#194490,#194491,#194492,#194493,
#194494,#194495,#194496,#194497,#194498,#194499,#194500,#194501,#194502,
#194503,#194504,#194505,#194506,#194507,#194508,#194509,#194510,#194511,
#194512,#194513,#194514,#194515,#194516,#194517,#194518,#194519,#194520,
#194521,#194522),.UNSPECIFIED.,.F.,.F.,(4,3,3,3,3,3,3,3,3,3,3,3,3,3,3,3,
3,4),(0.,4.29652152155444E-5,8.44519107519921E-5,0.000123669830862218,0.000159788877353411,
0.000170558847912627,0.000181218775907166,0.0001819600464524,0.000214460062643083,
0.00024475572619671,0.000255838271868938,0.000258503253867573,0.00026108495517875,
0.000289370476649592,0.000301101325502,0.000321109510663625,0.000331113603244437,
0.00034111769582525),.UNSPECIFIED.);
#4667=B_SPLINE_CURVE_WITH_KNOTS('',3,(#194524,#194525,#194526,#194527,#194528,
#194529,#194530,#194531,#194532,#194533,#194534,#194535,#194536,#194537,
#194538,#194539,#194540,#194541,#194542,#194543,#194544,#194545,#194546,
#194547,#194548,#194549,#194550,#194551,#194552,#194553,#194554,#194555,
#194556,#194557,#194558,#194559,#194560,#194561,#194562,#194563,#194564,
#194565,#194566,#194567,#194568,#194569,#194570,#194571,#194572,#194573,
#194574,#194575),.UNSPECIFIED.,.F.,.F.,(4,3,3,3,3,3,3,3,3,3,3,3,3,3,3,3,
3,4),(1.04083408558608E-17,4.30706237864328E-5,8.47417087688249E-5,0.000124159989204731,
0.000160467076288871,0.000170998382116696,0.00018241499473378,0.00021374797764587,
0.000242415955903496,0.000256497573175044,0.000259169422895617,0.000261757777312422,
0.000289965130403092,0.000301877270772907,0.000321937017503149,0.000326951954185709,
0.00033447435920955,0.000341996764233391),.UNSPECIFIED.);
#4668=B_SPLINE_CURVE_WITH_KNOTS('',3,(#194576,#194577,#194578,#194579,#194580,
#194581,#194582,#194583,#194584,#194585,#194586,#194587,#194588,#194589,
#194590,#194591,#194592,#194593,#194594,#194595,#194596,#194597,#194598,
#194599,#194600,#194601,#194602,#194603,#194604,#194605,#194606,#194607,
#194608,#194609,#194610,#194611,#194612,#194613,#194614,#194615,#194616,
#194617,#194618,#194619,#194620,#194621,#194622,#194623,#194624,#194625,
#194626,#194627),.UNSPECIFIED.,.F.,.F.,(4,3,3,3,3,3,3,3,3,3,3,3,3,3,3,3,
3,4),(1.73472347597681E-18,2.58457451674207E-5,4.25394446196043E-5,6.46659869687212E-5,
7.57292581432797E-5,8.12608937305589E-5,8.26438026273787E-5,8.67925293178381E-5,
0.000116015624426875,0.000130188793976756,0.000151886926306215,0.000161963651211264,
0.000162735992470945,0.000173585058635675,0.000212487880460368,0.000255238173510853,
0.000301397761146635,0.000347170117271375),.UNSPECIFIED.);
#4669=B_SPLINE_CURVE_WITH_KNOTS('',3,(#194629,#194630,#194631,#194632,#194633,
#194634,#194635,#194636,#194637,#194638,#194639,#194640,#194641,#194642,
#194643,#194644,#194645,#194646,#194647,#194648,#194649,#194650,#194651,
#194652,#194653,#194654,#194655,#194656,#194657,#194658,#194659,#194660,
#194661,#194662,#194663,#194664,#194665,#194666,#194667,#194668,#194669,
#194670,#194671,#194672,#194673,#194674),.UNSPECIFIED.,.F.,.F.,(4,3,3,3,
3,3,3,3,3,3,3,3,3,3,3,4),(0.,2.57218161994108E-5,4.21568322568941E-5,6.45873314617598E-5,
7.58025810641926E-5,8.14102058654091E-5,8.28121120657132E-5,8.70178306666255E-5,
0.000116081955658529,0.000130526745999938,0.000162394111022068,0.000174035661333251,
0.000213138396959093,0.000256116935435327,0.000302406662857997,0.000348071322666476),
 .UNSPECIFIED.);
#4670=B_SPLINE_CURVE_WITH_KNOTS('',3,(#194675,#194676,#194677,#194678,#194679,
#194680,#194681,#194682,#194683,#194684,#194685,#194686,#194687,#194688,
#194689,#194690,#194691,#194692,#194693,#194694,#194695,#194696,#194697,
#194698,#194699,#194700,#194701,#194702,#194703,#194704,#194705,#194706,
#194707,#194708,#194709,#194710,#194711,#194712,#194713,#194714,#194715,
#194716,#194717,#194718,#194719,#194720,#194721,#194722,#194723,#194724,
#194725,#194726),.UNSPECIFIED.,.F.,.F.,(4,3,3,3,3,3,3,3,3,3,3,3,3,3,3,3,
3,4),(0.,4.296521521763E-5,8.44519107554871E-5,0.000123669830866643,0.000159788877358575,
0.000170558847912618,0.000181218775907158,0.000181960046452402,0.000214460062644093,
0.00024475572619934,0.00025583827186894,0.000258503253867575,0.000261084955178753,
0.000289370476647943,0.000301101325502008,0.000321109510663635,0.000331113603244448,
0.000341117695825262),.UNSPECIFIED.);
#4671=B_SPLINE_CURVE_WITH_KNOTS('',3,(#194728,#194729,#194730,#194731,#194732,
#194733,#194734,#194735,#194736,#194737,#194738,#194739,#194740,#194741,
#194742,#194743,#194744,#194745,#194746,#194747,#194748,#194749,#194750,
#194751,#194752,#194753,#194754,#194755,#194756,#194757,#194758,#194759,
#194760,#194761,#194762,#194763,#194764,#194765,#194766,#194767,#194768,
#194769,#194770,#194771,#194772,#194773,#194774,#194775,#194776,#194777,
#194778,#194779),.UNSPECIFIED.,.F.,.F.,(4,3,3,3,3,3,3,3,3,3,3,3,3,3,3,3,
3,4),(9.96522768216898E-18,4.30706237863075E-5,8.47417087683585E-5,0.000124159989203683,
0.000160467076287053,0.000170998382116712,0.000182414994733787,0.000213747977645881,
0.000242415955903098,0.000256497573175051,0.000259169422895624,0.000261757777312429,
0.000289965130403181,0.000301877270772909,0.00032193701750315,0.00032695195418571,
0.00033447435920955,0.00034199676423339),.UNSPECIFIED.);
#4672=B_SPLINE_CURVE_WITH_KNOTS('',3,(#194780,#194781,#194782,#194783,#194784,
#194785,#194786,#194787,#194788,#194789,#194790,#194791,#194792,#194793,
#194794,#194795,#194796,#194797,#194798,#194799,#194800,#194801,#194802,
#194803,#194804,#194805,#194806,#194807,#194808,#194809,#194810,#194811,
#194812,#194813,#194814,#194815,#194816,#194817,#194818,#194819,#194820,
#194821,#194822,#194823,#194824,#194825,#194826,#194827,#194828,#194829,
#194830,#194831),.UNSPECIFIED.,.F.,.F.,(4,3,3,3,3,3,3,3,3,3,3,3,3,3,3,3,
3,4),(0.,2.58457451687118E-5,4.25394446195713E-5,6.46659869687085E-5,7.57292581432772E-5,
8.12608937305615E-5,8.26438026273826E-5,8.67925293178458E-5,0.000116015624427385,
0.000130188793976769,0.00015188692630623,0.000161963651211277,0.000162735992470961,
0.000173585058635692,0.000212487880461626,0.00025523817351366,0.000301397761151513,
0.000347170117271372),.UNSPECIFIED.);
#4673=B_SPLINE_CURVE_WITH_KNOTS('',3,(#194833,#194834,#194835,#194836,#194837,
#194838,#194839,#194840,#194841,#194842,#194843,#194844,#194845,#194846,
#194847,#194848,#194849,#194850,#194851,#194852,#194853,#194854,#194855,
#194856,#194857,#194858,#194859,#194860,#194861,#194862,#194863,#194864,
#194865,#194866,#194867,#194868,#194869,#194870,#194871,#194872,#194873,
#194874,#194875,#194876,#194877,#194878),.UNSPECIFIED.,.F.,.F.,(4,3,3,3,
3,3,3,3,3,3,3,3,3,3,3,4),(8.67361737988404E-19,2.57218161993721E-5,4.21568322568887E-5,
6.45873314617549E-5,7.5802581064188E-5,8.14102058654046E-5,8.28121120657087E-5,
8.70178306666211E-5,0.000116081955659502,0.000130526745999931,0.000162394111022061,
0.000174035661333241,0.000213138396957143,0.000256116935431465,0.000302406662852055,
0.000348071322666494),.UNSPECIFIED.);
#4674=B_SPLINE_CURVE_WITH_KNOTS('',3,(#194879,#194880,#194881,#194882,#194883,
#194884,#194885,#194886,#194887,#194888,#194889,#194890,#194891,#194892,
#194893,#194894,#194895,#194896,#194897,#194898,#194899,#194900,#194901,
#194902,#194903,#194904,#194905,#194906,#194907,#194908,#194909,#194910,
#194911,#194912,#194913,#194914,#194915,#194916,#194917,#194918,#194919,
#194920,#194921,#194922,#194923,#194924,#194925,#194926,#194927,#194928,
#194929,#194930),.UNSPECIFIED.,.F.,.F.,(4,3,3,3,3,3,3,3,3,3,3,3,3,3,3,3,
3,4),(0.,4.2965215213771E-5,8.44519107494884E-5,0.000123669830859856,0.000159788877351868,
0.000170558847912631,0.00018121877590717,0.000181960046452402,0.000214460062643814,
0.000244755726199141,0.000255838271868941,0.000258503253867576,0.000261084955178753,
0.000289370476648063,0.000301101325502002,0.000321109510663626,0.000331113603244439,
0.000341117695825251),.UNSPECIFIED.);
#4675=B_SPLINE_CURVE_WITH_KNOTS('',3,(#194932,#194933,#194934,#194935,#194936,
#194937,#194938,#194939,#194940,#194941,#194942,#194943,#194944,#194945,
#194946,#194947,#194948,#194949,#194950,#194951,#194952,#194953,#194954,
#194955,#194956,#194957,#194958,#194959,#194960,#194961,#194962,#194963,
#194964,#194965,#194966,#194967,#194968,#194969,#194970,#194971,#194972,
#194973,#194974,#194975,#194976,#194977,#194978,#194979,#194980,#194981,
#194982,#194983),.UNSPECIFIED.,.F.,.F.,(4,3,3,3,3,3,3,3,3,3,3,3,3,3,3,3,
3,4),(5.96311194867027E-19,4.30706237866237E-5,8.47417087690704E-5,0.0001241599892049,
0.000160467076288867,0.000170998382116678,0.000182414994733734,0.000213747977645854,
0.000242415955902605,0.00025649757317503,0.000259169422895604,0.000261757777312409,
0.000289965130403055,0.000301877270772896,0.000321937017503139,0.0003269519541857,
0.000334474359209541,0.000341996764233382),.UNSPECIFIED.);
#4676=B_SPLINE_CURVE_WITH_KNOTS('',3,(#194984,#194985,#194986,#194987,#194988,
#194989,#194990,#194991,#194992,#194993,#194994,#194995,#194996,#194997,
#194998,#194999,#195000,#195001,#195002,#195003,#195004,#195005,#195006,
#195007,#195008,#195009,#195010,#195011,#195012,#195013,#195014,#195015,
#195016,#195017,#195018,#195019,#195020,#195021,#195022,#195023,#195024,
#195025,#195026,#195027,#195028,#195029,#195030,#195031,#195032,#195033,
#195034,#195035),.UNSPECIFIED.,.F.,.F.,(4,3,3,3,3,3,3,3,3,3,3,3,3,3,3,3,
3,4),(0.,2.58457451671235E-5,4.25394446195251E-5,6.46659869686816E-5,7.57292581432598E-5,
8.12608937305489E-5,8.26438026273711E-5,8.6792529317838E-5,0.000116015624427186,
0.000130188793976757,0.000151886926306216,0.000161963651211284,0.000162735992470946,
0.000173585058635676,0.000212487880462066,0.000255238173513635,0.000301397761149358,
0.000347170117271353),.UNSPECIFIED.);
#4677=B_SPLINE_CURVE_WITH_KNOTS('',3,(#195037,#195038,#195039,#195040,#195041,
#195042,#195043,#195044,#195045,#195046,#195047,#195048,#195049,#195050,
#195051,#195052,#195053,#195054,#195055,#195056,#195057,#195058,#195059,
#195060,#195061,#195062,#195063,#195064,#195065,#195066,#195067,#195068,
#195069,#195070,#195071,#195072,#195073,#195074,#195075,#195076,#195077,
#195078,#195079,#195080,#195081,#195082),.UNSPECIFIED.,.F.,.F.,(4,3,3,3,
3,3,3,3,3,3,3,3,3,3,3,4),(2.74438674910393E-19,2.57218161990037E-5,4.21568322568875E-5,
6.45873314617528E-5,7.58025810641855E-5,8.14102058654018E-5,8.28121120657059E-5,
8.70178306666182E-5,0.000116081955659215,0.000130526745999927,0.000162394111022046,
0.000174035661333236,0.000213138396958664,0.000256116935434767,0.000302406662858074,
0.000348071322666484),.UNSPECIFIED.);
#4678=B_SPLINE_CURVE_WITH_KNOTS('',3,(#195083,#195084,#195085,#195086,#195087,
#195088,#195089,#195090,#195091,#195092,#195093,#195094,#195095,#195096,
#195097,#195098,#195099,#195100,#195101,#195102,#195103,#195104,#195105,
#195106,#195107,#195108,#195109,#195110,#195111,#195112,#195113,#195114,
#195115,#195116,#195117,#195118,#195119,#195120,#195121,#195122,#195123,
#195124,#195125,#195126,#195127,#195128,#195129,#195130,#195131,#195132,
#195133,#195134),.UNSPECIFIED.,.F.,.F.,(4,3,3,3,3,3,3,3,3,3,3,3,3,3,3,3,
3,4),(0.,4.29652152166783E-5,8.44519107543665E-5,0.000123669830866176,0.000159788877359447,
0.000170558847912639,0.000181218775907178,0.000181960046452414,0.000214460062643347,
0.000244755726197935,0.000255838271868953,0.000258503253867587,0.000261084955178765,
0.000289370476648123,0.000301101325502015,0.000321109510663641,0.000331113603244453,
0.000341117695825266),.UNSPECIFIED.);
#4679=B_SPLINE_CURVE_WITH_KNOTS('',3,(#195136,#195137,#195138,#195139,#195140,
#195141,#195142,#195143,#195144,#195145,#195146,#195147,#195148,#195149,
#195150,#195151,#195152,#195153,#195154,#195155,#195156,#195157,#195158,
#195159,#195160,#195161,#195162,#195163,#195164,#195165,#195166,#195167,
#195168,#195169,#195170,#195171,#195172,#195173,#195174,#195175,#195176,
#195177,#195178,#195179,#195180,#195181,#195182,#195183,#195184,#195185,
#195186,#195187),.UNSPECIFIED.,.F.,.F.,(4,3,3,3,3,3,3,3,3,3,3,3,3,3,3,3,
3,4),(0.,4.30706237874845E-5,8.47417087706428E-5,0.00012415998920723,0.000160467076292075,
0.000170998382116687,0.000182414994733767,0.000213747977645861,0.000242415955902588,
0.000256497573175036,0.000259169422895609,0.000261757777312415,0.000289965130404048,
0.0003018772707729,0.000321937017503143,0.000326951954185703,0.000334474359209544,
0.000341996764233385),.UNSPECIFIED.);
#4680=B_SPLINE_CURVE_WITH_KNOTS('',3,(#195188,#195189,#195190,#195191,#195192,
#195193,#195194,#195195,#195196,#195197,#195198,#195199,#195200,#195201,
#195202,#195203,#195204,#195205,#195206,#195207,#195208,#195209,#195210,
#195211,#195212,#195213,#195214,#195215,#195216,#195217,#195218,#195219,
#195220,#195221,#195222,#195223,#195224,#195225,#195226,#195227,#195228,
#195229,#195230,#195231,#195232,#195233,#195234,#195235,#195236,#195237,
#195238,#195239),.UNSPECIFIED.,.F.,.F.,(4,3,3,3,3,3,3,3,3,3,3,3,3,3,3,3,
3,4),(0.,2.58457451673457E-5,4.2539444619484E-5,6.46659869686634E-5,7.57292581432531E-5,
8.1260893730548E-5,8.26438026273717E-5,8.67925293178428E-5,0.000116015624427219,
0.000130188793976764,0.000151886926306225,0.000161963651211282,0.000162735992470955,
0.000173585058635686,0.000212487880462819,0.000255238173516115,0.000301397761155885,
0.000347170117271382),.UNSPECIFIED.);
#4681=B_SPLINE_CURVE_WITH_KNOTS('',3,(#195241,#195242,#195243,#195244,#195245,
#195246,#195247,#195248,#195249,#195250,#195251,#195252,#195253,#195254,
#195255,#195256,#195257,#195258,#195259,#195260,#195261,#195262,#195263,
#195264,#195265,#195266,#195267,#195268,#195269,#195270,#195271,#195272,
#195273,#195274,#195275,#195276,#195277,#195278,#195279,#195280,#195281,
#195282,#195283,#195284,#195285,#195286),.UNSPECIFIED.,.F.,.F.,(4,3,3,3,
3,3,3,3,3,3,3,3,3,3,3,4),(8.67361737988404E-19,2.57218161990736E-5,4.21568322568542E-5,
6.45873314617417E-5,7.58025810641855E-5,8.14102058654074E-5,8.28121120657128E-5,
8.70178306666293E-5,0.00011608195565874,0.000130526745999943,0.00016239411102208,
0.000174035661333258,0.000213138396959731,0.000256116935436739,0.000302406662860658,
0.000348071322666488),.UNSPECIFIED.);
#4682=B_SPLINE_CURVE_WITH_KNOTS('',3,(#195287,#195288,#195289,#195290,#195291,
#195292,#195293,#195294,#195295,#195296,#195297,#195298,#195299,#195300,
#195301,#195302,#195303,#195304,#195305,#195306,#195307,#195308,#195309,
#195310,#195311,#195312,#195313,#195314,#195315,#195316,#195317,#195318,
#195319,#195320,#195321,#195322,#195323,#195324,#195325,#195326,#195327,
#195328,#195329,#195330,#195331,#195332,#195333,#195334,#195335,#195336,
#195337,#195338),.UNSPECIFIED.,.F.,.F.,(4,3,3,3,3,3,3,3,3,3,3,3,3,3,3,3,
3,4),(0.,4.29652152202833E-5,8.44519107603119E-5,0.000123669830873692,0.000159788877368183,
0.000170558847912632,0.000181218775907171,0.000181960046452397,0.000214460062643704,
0.00024475572619857,0.000255838271868947,0.000258503253867581,0.000261084955178759,
0.000289370476647362,0.00030110132550201,0.000321109510663636,0.000331113603244449,
0.000341117695825261),.UNSPECIFIED.);
#4683=B_SPLINE_CURVE_WITH_KNOTS('',3,(#195340,#195341,#195342,#195343,#195344,
#195345,#195346,#195347,#195348,#195349,#195350,#195351,#195352,#195353,
#195354,#195355,#195356,#195357,#195358,#195359,#195360,#195361,#195362,
#195363,#195364,#195365,#195366,#195367,#195368,#195369,#195370,#195371,
#195372,#195373,#195374,#195375,#195376,#195377,#195378,#195379,#195380,
#195381,#195382,#195383,#195384,#195385,#195386,#195387,#195388,#195389,
#195390,#195391),.UNSPECIFIED.,.F.,.F.,(4,3,3,3,3,3,3,3,3,3,3,3,3,3,3,3,
3,4),(0.,4.30706237877163E-5,8.47417087709679E-5,0.000124159989207455,0.000160467076292245,
0.000170998382116692,0.000182414994733783,0.000213747977645868,0.000242415955903003,
0.000256497573175044,0.000259169422895617,0.000261757777312423,0.00028996513040353,
0.000301877270772909,0.000321937017503152,0.000326951954185713,0.000334474359209554,
0.000341996764233395),.UNSPECIFIED.);
#4684=B_SPLINE_CURVE_WITH_KNOTS('',3,(#195392,#195393,#195394,#195395,#195396,
#195397,#195398,#195399,#195400,#195401,#195402,#195403,#195404,#195405,
#195406,#195407,#195408,#195409,#195410,#195411,#195412,#195413,#195414,
#195415,#195416,#195417,#195418,#195419,#195420,#195421,#195422,#195423,
#195424,#195425,#195426,#195427,#195428,#195429,#195430,#195431,#195432,
#195433,#195434,#195435,#195436,#195437,#195438,#195439,#195440,#195441,
#195442,#195443),.UNSPECIFIED.,.F.,.F.,(4,3,3,3,3,3,3,3,3,3,3,3,3,3,3,3,
3,4),(0.,2.58457451689302E-5,4.25394446195954E-5,6.46659869687191E-5,7.57292581432809E-5,
8.12608937305618E-5,8.26438026273821E-5,8.67925293178427E-5,0.000116015624427155,
0.000130188793976764,0.000151886926306225,0.000161963651211299,0.000162735992470955,
0.000173585058635685,0.000212487880459557,0.000255238173508823,0.000301397761142415,
0.000347170117271368),.UNSPECIFIED.);
#4685=B_SPLINE_CURVE_WITH_KNOTS('',3,(#195445,#195446,#195447,#195448,#195449,
#195450,#195451,#195452,#195453,#195454,#195455,#195456,#195457,#195458,
#195459,#195460,#195461,#195462,#195463,#195464,#195465,#195466,#195467,
#195468,#195469,#195470,#195471,#195472,#195473,#195474,#195475,#195476,
#195477,#195478,#195479,#195480,#195481,#195482,#195483,#195484,#195485,
#195486,#195487,#195488,#195489,#195490),.UNSPECIFIED.,.F.,.F.,(4,3,3,3,
3,3,3,3,3,3,3,3,3,3,3,4),(0.,2.57218161989687E-5,4.21568322569323E-5,6.45873314617774E-5,
7.58025810641999E-5,8.14102058654112E-5,8.2812112065714E-5,8.70178306666224E-5,
0.000116081955658865,0.000130526745999934,0.000162394111022051,0.000174035661333245,
0.000213138396958673,0.000256116935434495,0.000302406662856898,0.000348071322666492),
 .UNSPECIFIED.);
#4686=B_SPLINE_CURVE_WITH_KNOTS('',3,(#195491,#195492,#195493,#195494,#195495,
#195496,#195497,#195498,#195499,#195500,#195501,#195502,#195503,#195504,
#195505,#195506,#195507,#195508,#195509,#195510,#195511,#195512,#195513,
#195514,#195515,#195516,#195517,#195518,#195519,#195520,#195521,#195522,
#195523,#195524,#195525,#195526,#195527,#195528,#195529,#195530,#195531,
#195532,#195533,#195534,#195535,#195536,#195537,#195538,#195539,#195540,
#195541,#195542),.UNSPECIFIED.,.F.,.F.,(4,3,3,3,3,3,3,3,3,3,3,3,3,3,3,3,
3,4),(0.,4.29652152166048E-5,8.44519107542708E-5,0.000123669830866133,0.000159788877359471,
0.000170558847912629,0.000181218775907169,0.000181960046452409,0.00021446006264399,
0.000244755726199507,0.000255838271868949,0.000258503253867584,0.000261084955178761,
0.000289370476647456,0.000301101325502015,0.000321109510663642,0.000331113603244455,
0.000341117695825268),.UNSPECIFIED.);
#4687=B_SPLINE_CURVE_WITH_KNOTS('',3,(#195544,#195545,#195546,#195547,#195548,
#195549,#195550,#195551,#195552,#195553,#195554,#195555,#195556,#195557,
#195558,#195559,#195560,#195561,#195562,#195563,#195564,#195565,#195566,
#195567,#195568,#195569,#195570,#195571,#195572,#195573,#195574,#195575,
#195576,#195577,#195578,#195579,#195580,#195581,#195582,#195583,#195584,
#195585,#195586,#195587,#195588,#195589,#195590,#195591,#195592,#195593,
#195594,#195595),.UNSPECIFIED.,.F.,.F.,(4,3,3,3,3,3,3,3,3,3,3,3,3,3,3,3,
3,4),(0.,4.30706237842305E-5,8.47417087646157E-5,0.000124159989198291,0.000160467076279865,
0.000170998382116677,0.000182414994733764,0.000213747977645854,0.000242415955901984,
0.000256497573175031,0.000259169422895605,0.000261757777312411,0.000289965130404686,
0.000301877270772898,0.000321937017503142,0.000326951954185703,0.000334474359209544,
0.000341996764233385),.UNSPECIFIED.);
#4688=B_SPLINE_CURVE_WITH_KNOTS('',3,(#195596,#195597,#195598,#195599,#195600,
#195601,#195602,#195603,#195604,#195605,#195606,#195607,#195608,#195609,
#195610,#195611,#195612,#195613,#195614,#195615,#195616,#195617,#195618,
#195619,#195620,#195621,#195622,#195623,#195624,#195625,#195626,#195627,
#195628,#195629,#195630,#195631,#195632,#195633,#195634,#195635,#195636,
#195637,#195638,#195639,#195640,#195641,#195642,#195643,#195644,#195645,
#195646,#195647),.UNSPECIFIED.,.F.,.F.,(4,3,3,3,3,3,3,3,3,3,3,3,3,3,3,3,
3,4),(3.46944695195361E-18,2.58457451680897E-5,4.25394446195799E-5,6.46659869687106E-5,
7.5729258143276E-5,8.12608937305587E-5,8.26438026273794E-5,8.67925293178414E-5,
0.000116015624427486,0.00013018879397676,0.00015188692630622,0.000161963651211284,
0.00016273599247095,0.000173585058635679,0.000212487880461467,0.00025523817351237,
0.000301397761147355,0.000347170117271362),.UNSPECIFIED.);
#4689=B_SPLINE_CURVE_WITH_KNOTS('',3,(#195649,#195650,#195651,#195652,#195653,
#195654,#195655,#195656,#195657,#195658,#195659,#195660,#195661,#195662,
#195663,#195664,#195665,#195666,#195667,#195668,#195669,#195670,#195671,
#195672,#195673,#195674,#195675,#195676,#195677,#195678,#195679,#195680,
#195681,#195682,#195683,#195684,#195685,#195686,#195687,#195688,#195689,
#195690,#195691,#195692,#195693,#195694),.UNSPECIFIED.,.F.,.F.,(4,3,3,3,
3,3,3,3,3,3,3,3,3,3,3,4),(0.,2.57218161988461E-5,4.21568322568433E-5,6.45873314617288E-5,
7.58025810641716E-5,8.1410205865393E-5,8.28121120656983E-5,8.70178306666144E-5,
0.00011608195565829,0.000130526745999922,0.000162394111022053,0.000174035661333229,
0.000213138396959319,0.000256116935436003,0.000302406662859732,0.00034807132266647),
 .UNSPECIFIED.);
#4690=B_SPLINE_CURVE_WITH_KNOTS('',3,(#195695,#195696,#195697,#195698,#195699,
#195700,#195701,#195702,#195703,#195704,#195705,#195706,#195707,#195708,
#195709,#195710,#195711,#195712,#195713,#195714,#195715,#195716,#195717,
#195718,#195719,#195720,#195721,#195722,#195723,#195724,#195725,#195726,
#195727,#195728,#195729,#195730,#195731,#195732,#195733,#195734,#195735,
#195736,#195737,#195738,#195739,#195740,#195741,#195742,#195743,#195744,
#195745,#195746),.UNSPECIFIED.,.F.,.F.,(4,3,3,3,3,3,3,3,3,3,3,3,3,3,3,3,
3,4),(0.,4.29652152158802E-5,8.44519107530096E-5,0.000123669830864391,0.000159788877357164,
0.000170558847912637,0.000181218775907177,0.000181960046452427,0.000214460062643589,
0.000244755726198111,0.000255838271868954,0.000258503253867589,0.000261084955178767,
0.000289370476648303,0.000301101325502019,0.000321109510663645,0.000331113603244458,
0.000341117695825271),.UNSPECIFIED.);
#4691=B_SPLINE_CURVE_WITH_KNOTS('',3,(#195748,#195749,#195750,#195751,#195752,
#195753,#195754,#195755,#195756,#195757,#195758,#195759,#195760,#195761,
#195762,#195763,#195764,#195765,#195766,#195767,#195768,#195769,#195770,
#195771,#195772,#195773,#195774,#195775,#195776,#195777,#195778,#195779,
#195780,#195781,#195782,#195783,#195784,#195785,#195786,#195787,#195788,
#195789,#195790,#195791,#195792,#195793,#195794,#195795,#195796,#195797,
#195798,#195799),.UNSPECIFIED.,.F.,.F.,(4,3,3,3,3,3,3,3,3,3,3,3,3,3,3,3,
3,4),(0.,4.30706237886451E-5,8.4741708772696E-5,0.000124159989209975,0.0001604670762956,
0.000170998382116695,0.000182414994733774,0.000213747977645868,0.000242415955903289,
0.000256497573175042,0.000259169422895615,0.00026175777731242,0.000289965130403147,
0.000301877270772904,0.000321937017503146,0.000326951954185707,0.000334474359209547,
0.000341996764233388),.UNSPECIFIED.);
#4692=B_SPLINE_CURVE_WITH_KNOTS('',3,(#195800,#195801,#195802,#195803,#195804,
#195805,#195806,#195807,#195808,#195809,#195810,#195811,#195812,#195813,
#195814,#195815,#195816,#195817,#195818,#195819,#195820,#195821,#195822,
#195823,#195824,#195825,#195826,#195827,#195828,#195829,#195830,#195831,
#195832,#195833,#195834,#195835,#195836,#195837,#195838,#195839,#195840,
#195841,#195842,#195843,#195844,#195845,#195846,#195847,#195848,#195849,
#195850,#195851),.UNSPECIFIED.,.F.,.F.,(4,3,3,3,3,3,3,3,3,3,3,3,3,3,3,3,
3,4),(0.,2.58457451684994E-5,4.25394446194796E-5,6.466598696866E-5,7.57292581432503E-5,
8.12608937305454E-5,8.26438026273691E-5,8.67925293178405E-5,0.000116015624427484,
0.000130188793976761,0.000151886926306221,0.000161963651211264,0.000162735992470951,
0.000173585058635681,0.000212487880461759,0.000255238173513016,0.000301397761148625,
0.000347170117271374),.UNSPECIFIED.);
#4693=B_SPLINE_CURVE_WITH_KNOTS('',3,(#195853,#195854,#195855,#195856,#195857,
#195858,#195859,#195860,#195861,#195862,#195863,#195864,#195865,#195866,
#195867,#195868,#195869,#195870,#195871,#195872,#195873,#195874,#195875,
#195876,#195877,#195878,#195879,#195880,#195881,#195882,#195883,#195884,
#195885,#195886,#195887,#195888,#195889,#195890,#195891,#195892,#195893,
#195894,#195895,#195896,#195897,#195898),.UNSPECIFIED.,.F.,.F.,(4,3,3,3,
3,3,3,3,3,3,3,3,3,3,3,4),(0.,2.57218162002198E-5,4.21568322567467E-5,6.45873314616841E-5,
7.58025810641528E-5,8.14102058653871E-5,8.28121120656957E-5,8.70178306666214E-5,
0.000116081955658617,0.000130526745999932,0.000162394111022051,0.000174035661333243,
0.000213138396957433,0.000256116935432043,0.000302406662852999,0.000348071322666481),
 .UNSPECIFIED.);
#4694=B_SPLINE_CURVE_WITH_KNOTS('',3,(#195899,#195900,#195901,#195902,#195903,
#195904,#195905,#195906,#195907,#195908,#195909,#195910,#195911,#195912,
#195913,#195914,#195915,#195916,#195917,#195918,#195919,#195920,#195921,
#195922,#195923,#195924,#195925,#195926,#195927,#195928,#195929,#195930,
#195931,#195932,#195933,#195934,#195935,#195936,#195937,#195938,#195939,
#195940,#195941,#195942,#195943,#195944,#195945,#195946,#195947,#195948,
#195949,#195950),.UNSPECIFIED.,.F.,.F.,(4,3,3,3,3,3,3,3,3,3,3,3,3,3,3,3,
3,4),(0.,4.29652152173429E-5,8.44519107554398E-5,0.000123669830867436,0.00015978887736076,
0.000170558847912635,0.000181218775907174,0.000181960046452407,0.000214460062643482,
0.000244755726198295,0.000255838271868951,0.000258503253867586,0.000261084955178764,
0.000289370476647682,0.000301101325502016,0.000321109510663642,0.000331113603244455,
0.000341117695825268),.UNSPECIFIED.);
#4695=B_SPLINE_CURVE_WITH_KNOTS('',3,(#195952,#195953,#195954,#195955,#195956,
#195957,#195958,#195959,#195960,#195961,#195962,#195963,#195964,#195965,
#195966,#195967,#195968,#195969,#195970,#195971,#195972,#195973,#195974,
#195975,#195976,#195977,#195978,#195979,#195980,#195981,#195982,#195983,
#195984,#195985,#195986,#195987,#195988,#195989,#195990,#195991,#195992,
#195993,#195994,#195995,#195996,#195997,#195998,#195999,#196000,#196001,
#196002,#196003),.UNSPECIFIED.,.F.,.F.,(4,3,3,3,3,3,3,3,3,3,3,3,3,3,3,3,
3,4),(0.,4.30706237823169E-5,8.47417087612841E-5,0.000124159989193728,0.000160467076274024,
0.00017099838211669,0.000182414994733806,0.000213747977645865,0.000242415955902471,
0.000256497573175041,0.000259169422895614,0.00026175777731242,0.000289965130404446,
0.000301877270772906,0.000321937017503149,0.000326951954185709,0.00033447435920955,
0.000341996764233392),.UNSPECIFIED.);
#4696=B_SPLINE_CURVE_WITH_KNOTS('',3,(#196004,#196005,#196006,#196007,#196008,
#196009,#196010,#196011,#196012,#196013,#196014,#196015,#196016,#196017,
#196018,#196019,#196020,#196021,#196022,#196023,#196024,#196025,#196026,
#196027,#196028,#196029,#196030,#196031,#196032,#196033,#196034,#196035,
#196036,#196037,#196038,#196039,#196040,#196041,#196042,#196043,#196044,
#196045,#196046,#196047,#196048,#196049,#196050,#196051,#196052,#196053,
#196054,#196055),.UNSPECIFIED.,.F.,.F.,(4,3,3,3,3,3,3,3,3,3,3,3,3,3,3,3,
3,4),(0.,2.58457451671982E-5,4.25394446196549E-5,6.4665986968747E-5,7.5729258143293E-5,
8.12608937305661E-5,8.26438026273843E-5,8.67925293178391E-5,0.00011601562442746,
0.000130188793976759,0.000151886926306218,0.000161963651211268,0.000162735992470948,
0.000173585058635678,0.000212487880462689,0.000255238173515773,0.00030139776115473,
0.000347170117271358),.UNSPECIFIED.);
#4697=B_SPLINE_CURVE_WITH_KNOTS('',3,(#196057,#196058,#196059,#196060,#196061,
#196062,#196063,#196064,#196065,#196066,#196067,#196068,#196069,#196070,
#196071,#196072,#196073,#196074,#196075,#196076,#196077,#196078,#196079,
#196080,#196081,#196082,#196083,#196084,#196085,#196086,#196087,#196088,
#196089,#196090,#196091,#196092,#196093,#196094,#196095,#196096,#196097,
#196098,#196099,#196100,#196101,#196102),.UNSPECIFIED.,.F.,.F.,(4,3,3,3,
3,3,3,3,3,3,3,3,3,3,3,4),(0.,2.57218162004827E-5,4.21568322567461E-5,6.4587331461682E-5,
7.58025810641499E-5,8.14102058653839E-5,8.28121120656924E-5,8.70178306666178E-5,
0.000116081955659027,0.000130526745999927,0.000162394111022054,0.000174035661333236,
0.00021313839695725,0.000256116935432016,0.000302406662854051,0.000348071322666459),
 .UNSPECIFIED.);
#4698=B_SPLINE_CURVE_WITH_KNOTS('',3,(#196103,#196104,#196105,#196106,#196107,
#196108,#196109,#196110,#196111,#196112,#196113,#196114,#196115,#196116,
#196117,#196118,#196119,#196120,#196121,#196122,#196123,#196124,#196125,
#196126,#196127,#196128,#196129,#196130,#196131,#196132,#196133,#196134,
#196135,#196136,#196137,#196138,#196139,#196140,#196141,#196142,#196143,
#196144,#196145,#196146,#196147,#196148,#196149,#196150,#196151,#196152,
#196153,#196154),.UNSPECIFIED.,.F.,.F.,(4,3,3,3,3,3,3,3,3,3,3,3,3,3,3,3,
3,4),(0.,4.29652152210268E-5,8.44519107616881E-5,0.000123669830875786,0.000159788877371095,
0.000170558847912614,0.000181218775907154,0.0001819600464524,0.000214460062643448,
0.000244755726197702,0.000255838271868935,0.00025850325386757,0.000261084955178747,
0.000289370476647446,0.000301101325502001,0.000321109510663628,0.000331113603244442,
0.000341117695825255),.UNSPECIFIED.);
#4699=B_SPLINE_CURVE_WITH_KNOTS('',3,(#196156,#196157,#196158,#196159,#196160,
#196161,#196162,#196163,#196164,#196165,#196166,#196167,#196168,#196169,
#196170,#196171,#196172,#196173,#196174,#196175,#196176,#196177,#196178,
#196179,#196180,#196181,#196182,#196183,#196184,#196185,#196186,#196187,
#196188,#196189,#196190,#196191,#196192,#196193,#196194,#196195,#196196,
#196197,#196198,#196199,#196200,#196201,#196202,#196203,#196204,#196205,
#196206,#196207),.UNSPECIFIED.,.F.,.F.,(4,3,3,3,3,3,3,3,3,3,3,3,3,3,3,3,
3,4),(0.,4.30706237873732E-5,8.47417087705962E-5,0.000124159989207352,0.000160467076292369,
0.000170998382116696,0.000182414994733765,0.000213747977645869,0.000242415955903072,
0.000256497573175042,0.000259169422895615,0.000261757777312421,0.000289965130403374,
0.000301877270772904,0.000321937017503146,0.000326951954185707,0.000334474359209547,
0.000341996764233388),.UNSPECIFIED.);
#4700=B_SPLINE_CURVE_WITH_KNOTS('',3,(#196208,#196209,#196210,#196211,#196212,
#196213,#196214,#196215,#196216,#196217,#196218,#196219,#196220,#196221,
#196222,#196223,#196224,#196225,#196226,#196227,#196228,#196229,#196230,
#196231,#196232,#196233,#196234,#196235,#196236,#196237,#196238,#196239,
#196240,#196241,#196242,#196243,#196244,#196245,#196246,#196247,#196248,
#196249,#196250,#196251,#196252,#196253,#196254,#196255,#196256,#196257,
#196258,#196259),.UNSPECIFIED.,.F.,.F.,(4,3,3,3,3,3,3,3,3,3,3,3,3,3,3,3,
3,4),(0.,2.58457451703126E-5,4.25394446196281E-5,6.46659869687304E-5,7.57292581432815E-5,
8.12608937305571E-5,8.2643802627376E-5,8.67925293178326E-5,0.000116015624428797,
0.000130188793976749,0.000151886926306207,0.000161963651211271,0.000162735992470936,
0.000173585058635665,0.000212487880461566,0.000255238173512672,0.000301397761147969,
0.000347170117271347),.UNSPECIFIED.);
#4701=B_SPLINE_CURVE_WITH_KNOTS('',3,(#196261,#196262,#196263,#196264,#196265,
#196266,#196267,#196268,#196269,#196270,#196271,#196272,#196273,#196274,
#196275,#196276,#196277,#196278,#196279,#196280,#196281,#196282,#196283,
#196284,#196285,#196286,#196287,#196288,#196289,#196290,#196291,#196292,
#196293,#196294,#196295,#196296,#196297,#196298,#196299,#196300,#196301,
#196302,#196303,#196304,#196305,#196306),.UNSPECIFIED.,.F.,.F.,(4,3,3,3,
3,3,3,3,3,3,3,3,3,3,3,4),(0.,2.57218161992659E-5,4.21568322566835E-5,6.45873314616532E-5,
7.58025810641381E-5,8.14102058653805E-5,8.28121120656911E-5,8.70178306666229E-5,
0.00011608195565876,0.000130526745999934,0.000162394111022074,0.000174035661333246,
0.00021313839696108,0.000256116935439352,0.000302406662864497,0.000348071322666474),
 .UNSPECIFIED.);
#4702=B_SPLINE_CURVE_WITH_KNOTS('',3,(#196307,#196308,#196309,#196310,#196311,
#196312,#196313,#196314,#196315,#196316,#196317,#196318,#196319,#196320,
#196321,#196322,#196323,#196324,#196325,#196326,#196327,#196328,#196329,
#196330,#196331,#196332,#196333,#196334,#196335,#196336,#196337,#196338,
#196339,#196340,#196341,#196342,#196343,#196344,#196345,#196346,#196347,
#196348,#196349,#196350,#196351,#196352,#196353,#196354,#196355,#196356,
#196357,#196358),.UNSPECIFIED.,.F.,.F.,(4,3,3,3,3,3,3,3,3,3,3,3,3,3,3,3,
3,4),(0.,4.29652152199114E-5,8.44519107592339E-5,0.000123669830871405,0.000159788877364126,
0.000170558847912617,0.000181218775907156,0.000181960046452403,0.000214460062642956,
0.000244755726197005,0.000255838271868931,0.000258503253867566,0.000261084955178744,
0.000289370476649217,0.000301101325501995,0.00032110951066362,0.000331113603244433,
0.000341117695825246),.UNSPECIFIED.);
#4703=B_SPLINE_CURVE_WITH_KNOTS('',3,(#196360,#196361,#196362,#196363,#196364,
#196365,#196366,#196367,#196368,#196369,#196370,#196371,#196372,#196373,
#196374,#196375,#196376,#196377,#196378,#196379,#196380,#196381,#196382,
#196383,#196384,#196385,#196386,#196387,#196388,#196389,#196390,#196391,
#196392,#196393,#196394,#196395,#196396,#196397,#196398,#196399,#196400,
#196401,#196402,#196403,#196404,#196405,#196406,#196407,#196408,#196409,
#196410,#196411),.UNSPECIFIED.,.F.,.F.,(4,3,3,3,3,3,3,3,3,3,3,3,3,3,3,3,
3,4),(0.,4.30706237903638E-5,8.47417087757578E-5,0.000124159989214328,0.000160467076301428,
0.000170998382116691,0.000182414994733775,0.000213747977645864,0.000242415955904961,
0.000256497573175038,0.000259169422895611,0.000261757777312417,0.00028996513040181,
0.000301877270772901,0.000321937017503143,0.000326951954185704,0.000334474359209545,
0.000341996764233386),.UNSPECIFIED.);
#4704=B_SPLINE_CURVE_WITH_KNOTS('',3,(#196412,#196413,#196414,#196415,#196416,
#196417,#196418,#196419,#196420,#196421,#196422,#196423,#196424,#196425,
#196426,#196427,#196428,#196429,#196430,#196431,#196432,#196433,#196434,
#196435,#196436,#196437,#196438,#196439,#196440,#196441,#196442,#196443,
#196444,#196445,#196446,#196447,#196448,#196449,#196450,#196451,#196452,
#196453,#196454,#196455,#196456,#196457,#196458,#196459,#196460,#196461,
#196462,#196463),.UNSPECIFIED.,.F.,.F.,(4,3,3,3,3,3,3,3,3,3,3,3,3,3,3,3,
3,4),(0.,2.58457451685466E-5,4.25394446196209E-5,6.46659869687306E-5,7.57292581432855E-5,
8.12608937305629E-5,8.26438026273823E-5,8.67925293178403E-5,0.000116015624427434,
0.00013018879397676,0.000151886926306221,0.000161963651211266,0.000162735992470951,
0.000173585058635681,0.000212487880459847,0.000255238173510006,0.000301397761145795,
0.000347170117271344),.UNSPECIFIED.);
#4705=B_SPLINE_CURVE_WITH_KNOTS('',3,(#196465,#196466,#196467,#196468,#196469,
#196470,#196471,#196472,#196473,#196474,#196475,#196476,#196477,#196478,
#196479,#196480,#196481,#196482,#196483,#196484,#196485,#196486,#196487,
#196488,#196489,#196490,#196491,#196492,#196493,#196494,#196495,#196496,
#196497,#196498,#196499,#196500,#196501,#196502,#196503,#196504,#196505,
#196506,#196507,#196508,#196509,#196510),.UNSPECIFIED.,.F.,.F.,(4,3,3,3,
3,3,3,3,3,3,3,3,3,3,3,4),(0.,2.57218162017772E-5,4.21568322567134E-5,6.4587331461665E-5,
7.58025810641408E-5,8.14102058653787E-5,8.28121120656881E-5,8.70178306666165E-5,
0.000116081955658973,0.000130526745999925,0.000162394111022045,0.000174035661333233,
0.000213138396960719,0.000256116935438802,0.00030240666286413,0.000348071322666467),
 .UNSPECIFIED.);
#4706=B_SPLINE_CURVE_WITH_KNOTS('',3,(#196511,#196512,#196513,#196514,#196515,
#196516,#196517,#196518,#196519,#196520,#196521,#196522,#196523,#196524,
#196525,#196526,#196527,#196528,#196529,#196530,#196531,#196532,#196533,
#196534,#196535,#196536,#196537,#196538,#196539,#196540,#196541,#196542,
#196543,#196544,#196545,#196546,#196547,#196548,#196549,#196550,#196551,
#196552,#196553,#196554,#196555,#196556,#196557,#196558,#196559,#196560,
#196561,#196562),.UNSPECIFIED.,.F.,.F.,(4,3,3,3,3,3,3,3,3,3,3,3,3,3,3,3,
3,4),(0.,4.29652152161511E-5,8.4451910753523E-5,0.000123669830865121,0.000159788877358086,
0.000170558847912621,0.000181218775907161,0.000181960046452392,0.000214460062644014,
0.000244755726199354,0.000255838271868946,0.000258503253867581,0.000261084955178759,
0.000289370476646352,0.000301101325502015,0.000321109510663643,0.000331113603244457,
0.000341117695825271),.UNSPECIFIED.);
#4707=B_SPLINE_CURVE_WITH_KNOTS('',3,(#196564,#196565,#196566,#196567,#196568,
#196569,#196570,#196571,#196572,#196573,#196574,#196575,#196576,#196577,
#196578,#196579,#196580,#196581,#196582,#196583,#196584,#196585,#196586,
#196587,#196588,#196589,#196590,#196591,#196592,#196593,#196594,#196595,
#196596,#196597,#196598,#196599,#196600,#196601,#196602,#196603,#196604,
#196605,#196606,#196607,#196608,#196609,#196610,#196611,#196612,#196613,
#196614,#196615),.UNSPECIFIED.,.F.,.F.,(4,3,3,3,3,3,3,3,3,3,3,3,3,3,3,3,
3,4),(0.,4.30706237866705E-5,8.47417087691936E-5,0.000124159989205159,0.000160467076289346,
0.000170998382116694,0.000182414994733781,0.000213747977645868,0.000242415955904174,
0.000256497573175041,0.000259169422895614,0.00026175777731242,0.000289965130405258,
0.000301877270772903,0.000321937017503145,0.000326951954185706,0.000334474359209547,
0.000341996764233387),.UNSPECIFIED.);
#4708=B_SPLINE_CURVE_WITH_KNOTS('',3,(#196616,#196617,#196618,#196619,#196620,
#196621,#196622,#196623,#196624,#196625,#196626,#196627,#196628,#196629,
#196630,#196631,#196632,#196633,#196634,#196635,#196636,#196637,#196638,
#196639,#196640,#196641,#196642,#196643,#196644,#196645,#196646,#196647,
#196648,#196649,#196650,#196651,#196652,#196653,#196654,#196655,#196656,
#196657,#196658,#196659,#196660,#196661,#196662,#196663,#196664,#196665,
#196666,#196667),.UNSPECIFIED.,.F.,.F.,(4,3,3,3,3,3,3,3,3,3,3,3,3,3,3,3,
3,4),(0.,2.58457451669911E-5,4.25394446195997E-5,6.46659869687207E-5,7.57292581432812E-5,
8.12608937305615E-5,8.26438026273815E-5,8.67925293178417E-5,0.000116015624426113,
0.000130188793976763,0.000151886926306223,0.000161963651211266,0.000162735992470953,
0.000173585058635683,0.000212487880456845,0.000255238173501831,0.000301397761127879,
0.00034717011727138),.UNSPECIFIED.);
#4709=B_SPLINE_CURVE_WITH_KNOTS('',3,(#196669,#196670,#196671,#196672,#196673,
#196674,#196675,#196676,#196677,#196678,#196679,#196680,#196681,#196682,
#196683,#196684,#196685,#196686,#196687,#196688,#196689,#196690,#196691,
#196692,#196693,#196694,#196695,#196696,#196697,#196698,#196699,#196700,
#196701,#196702,#196703,#196704,#196705,#196706,#196707,#196708,#196709,
#196710,#196711,#196712,#196713,#196714),.UNSPECIFIED.,.F.,.F.,(4,3,3,3,
3,3,3,3,3,3,3,3,3,3,3,4),(0.,2.57218161991998E-5,4.21568322567933E-5,6.45873314617068E-5,
7.58025810641636E-5,8.14102058653919E-5,8.2812112065699E-5,8.70178306666203E-5,
0.000116081955658395,0.00013052674599993,0.000162394111022055,0.000174035661333241,
0.000213138396959329,0.000256116935435947,0.000302406662859352,0.00034807132266647),
 .UNSPECIFIED.);
#4710=B_SPLINE_CURVE_WITH_KNOTS('',3,(#196715,#196716,#196717,#196718,#196719,
#196720,#196721,#196722,#196723,#196724,#196725,#196726,#196727,#196728,
#196729,#196730,#196731,#196732,#196733,#196734,#196735,#196736,#196737,
#196738,#196739,#196740,#196741,#196742,#196743,#196744,#196745,#196746,
#196747,#196748,#196749,#196750,#196751,#196752,#196753,#196754,#196755,
#196756,#196757,#196758,#196759,#196760,#196761,#196762,#196763,#196764,
#196765,#196766),.UNSPECIFIED.,.F.,.F.,(4,3,3,3,3,3,3,3,3,3,3,3,3,3,3,3,
3,4),(0.,4.29652152145126E-5,8.44519107508585E-5,0.000123669830861906,0.0001597888773547,
0.000170558847912636,0.000181218775907175,0.000181960046452407,0.000214460062643629,
0.000244755726198551,0.000255838271868953,0.000258503253867588,0.000261084955178766,
0.000289370476648523,0.000301101325502018,0.000321109510663644,0.000331113603244457,
0.00034111769582527),.UNSPECIFIED.);
#4711=B_SPLINE_CURVE_WITH_KNOTS('',3,(#196768,#196769,#196770,#196771,#196772,
#196773,#196774,#196775,#196776,#196777,#196778,#196779,#196780,#196781,
#196782,#196783,#196784,#196785,#196786,#196787,#196788,#196789,#196790,
#196791,#196792,#196793,#196794,#196795,#196796,#196797,#196798,#196799,
#196800,#196801,#196802,#196803,#196804,#196805,#196806,#196807,#196808,
#196809,#196810,#196811,#196812,#196813,#196814,#196815,#196816,#196817,
#196818,#196819),.UNSPECIFIED.,.F.,.F.,(4,3,3,3,3,3,3,3,3,3,3,3,3,3,3,3,
3,4),(0.,4.30706237893538E-5,8.47417087739242E-5,0.000124159989211692,0.000160467076297654,
0.0001709983821167,0.000182414994733784,0.000213747977645873,0.000242415955902547,
0.000256497573175046,0.000259169422895619,0.000261757777312425,0.000289965130402395,
0.000301877270772908,0.00032193701750315,0.000326951954185711,0.000334474359209551,
0.000341996764233392),.UNSPECIFIED.);
#4712=B_SPLINE_CURVE_WITH_KNOTS('',3,(#196820,#196821,#196822,#196823,#196824,
#196825,#196826,#196827,#196828,#196829,#196830,#196831,#196832,#196833,
#196834,#196835,#196836,#196837,#196838,#196839,#196840,#196841,#196842,
#196843,#196844,#196845,#196846,#196847,#196848,#196849,#196850,#196851,
#196852,#196853,#196854,#196855,#196856,#196857,#196858,#196859,#196860,
#196861,#196862,#196863,#196864,#196865,#196866,#196867,#196868,#196869,
#196870,#196871),.UNSPECIFIED.,.F.,.F.,(4,3,3,3,3,3,3,3,3,3,3,3,3,3,3,3,
3,4),(0.,2.58457451681646E-5,4.25394446194625E-5,6.46659869686492E-5,7.57292581432425E-5,
8.12608937305392E-5,8.26438026273634E-5,8.67925293178359E-5,0.000116015624428639,
0.000130188793976754,0.000151886926306213,0.000161963651211277,0.000162735992470942,
0.000173585058635672,0.000212487880460382,0.00025523817351074,0.000301397761146053,
0.00034717011727136),.UNSPECIFIED.);
#4713=B_SPLINE_CURVE_WITH_KNOTS('',3,(#196873,#196874,#196875,#196876,#196877,
#196878,#196879,#196880,#196881,#196882,#196883,#196884,#196885,#196886,
#196887,#196888,#196889,#196890,#196891,#196892,#196893,#196894,#196895,
#196896,#196897,#196898,#196899,#196900,#196901,#196902,#196903,#196904,
#196905,#196906,#196907,#196908,#196909,#196910,#196911,#196912,#196913,
#196914,#196915,#196916,#196917,#196918),.UNSPECIFIED.,.F.,.F.,(4,3,3,3,
3,3,3,3,3,3,3,3,3,3,3,4),(6.93889390390723E-18,2.57218162012745E-5,4.21568322568842E-5,
6.45873314617536E-5,7.58025810641882E-5,8.14102058654056E-5,8.28121120657099E-5,
8.70178306666229E-5,0.000116081955657485,0.000130526745999931,0.000162394111022046,
0.000174035661333239,0.000213138396958867,0.000256116935434972,0.000302406662857771,
0.000348071322666458),.UNSPECIFIED.);
#4714=B_SPLINE_CURVE_WITH_KNOTS('',3,(#196919,#196920,#196921,#196922,#196923,
#196924,#196925,#196926,#196927,#196928,#196929,#196930,#196931,#196932,
#196933,#196934,#196935,#196936,#196937,#196938,#196939,#196940,#196941,
#196942,#196943,#196944,#196945,#196946,#196947,#196948,#196949,#196950,
#196951,#196952,#196953,#196954,#196955,#196956,#196957,#196958,#196959,
#196960,#196961,#196962,#196963,#196964,#196965,#196966,#196967,#196968,
#196969,#196970),.UNSPECIFIED.,.F.,.F.,(4,3,3,3,3,3,3,3,3,3,3,3,3,3,3,3,
3,4),(0.,4.29652152149597E-5,8.4451910751605E-5,0.000123669830862903,0.000159788877355898,
0.000170558847912635,0.000181218775907175,0.000181960046452407,0.000214460062643025,
0.00024475572619701,0.000255838271868953,0.000258503253867588,0.000261084955178765,
0.000289370476648861,0.000301101325502018,0.000321109510663644,0.000331113603244457,
0.00034111769582527),.UNSPECIFIED.);
#4715=B_SPLINE_CURVE_WITH_KNOTS('',3,(#196972,#196973,#196974,#196975,#196976,
#196977,#196978,#196979,#196980,#196981,#196982,#196983,#196984,#196985,
#196986,#196987,#196988,#196989,#196990,#196991,#196992,#196993,#196994,
#196995,#196996,#196997,#196998,#196999,#197000,#197001,#197002,#197003,
#197004,#197005,#197006,#197007,#197008,#197009,#197010,#197011,#197012,
#197013,#197014,#197015,#197016,#197017,#197018,#197019,#197020,#197021,
#197022,#197023),.UNSPECIFIED.,.F.,.F.,(4,3,3,3,3,3,3,3,3,3,3,3,3,3,3,3,
3,4),(0.,4.30706237845979E-5,8.4741708765375E-5,0.00012415998919943,0.00016046707628152,
0.00017099838211669,0.000182414994733782,0.000213747977645867,0.000242415955903715,
0.000256497573175044,0.000259169422895618,0.000261757777312424,0.000289965130403571,
0.000301877270772911,0.000321937017503155,0.000326951954185716,0.000334474359209558,
0.000341996764233399),.UNSPECIFIED.);
#4716=B_SPLINE_CURVE_WITH_KNOTS('',3,(#197024,#197025,#197026,#197027,#197028,
#197029,#197030,#197031,#197032,#197033,#197034,#197035,#197036,#197037,
#197038,#197039,#197040,#197041,#197042,#197043,#197044,#197045,#197046,
#197047,#197048,#197049,#197050,#197051,#197052,#197053,#197054,#197055,
#197056,#197057,#197058,#197059,#197060,#197061,#197062,#197063,#197064,
#197065,#197066,#197067,#197068,#197069,#197070,#197071,#197072,#197073,
#197074,#197075),.UNSPECIFIED.,.F.,.F.,(4,3,3,3,3,3,3,3,3,3,3,3,3,3,3,3,
3,4),(3.46944695195361E-18,2.58457451685079E-5,4.25394446195536E-5,6.46659869686988E-5,
7.57292581432714E-5,8.12608937305577E-5,8.26438026273792E-5,8.6792529317844E-5,
0.000116015624427737,0.000130188793976764,0.000151886926306224,0.000161963651211275,
0.000162735992470954,0.000173585058635684,0.000212487880460469,0.000255238173510927,
0.00030139776114628,0.000347170117271379),.UNSPECIFIED.);
#4717=B_SPLINE_CURVE_WITH_KNOTS('',3,(#197077,#197078,#197079,#197080,#197081,
#197082,#197083,#197084,#197085,#197086,#197087,#197088,#197089,#197090,
#197091,#197092,#197093,#197094,#197095,#197096,#197097,#197098,#197099,
#197100,#197101,#197102,#197103,#197104,#197105,#197106,#197107,#197108,
#197109,#197110,#197111,#197112,#197113,#197114,#197115,#197116,#197117,
#197118,#197119,#197120,#197121,#197122),.UNSPECIFIED.,.F.,.F.,(4,3,3,3,
3,3,3,3,3,3,3,3,3,3,3,4),(0.,2.57218161989107E-5,4.21568322568349E-5,6.45873314617258E-5,
7.58025810641712E-5,8.1410205865394E-5,8.28121120656996E-5,8.70178306666167E-5,
0.000116081955658387,0.000130526745999925,0.00016239411102205,0.000174035661333233,
0.000213138396959998,0.000256116935437306,0.0003024066628616,0.000348071322666454),
 .UNSPECIFIED.);
#4718=B_SPLINE_CURVE_WITH_KNOTS('',3,(#197123,#197124,#197125,#197126,#197127,
#197128,#197129,#197130,#197131,#197132,#197133,#197134,#197135,#197136,
#197137,#197138,#197139,#197140,#197141,#197142,#197143,#197144,#197145,
#197146,#197147,#197148,#197149,#197150,#197151,#197152,#197153,#197154,
#197155,#197156,#197157,#197158,#197159,#197160,#197161,#197162,#197163,
#197164,#197165,#197166,#197167,#197168,#197169,#197170,#197171,#197172,
#197173,#197174),.UNSPECIFIED.,.F.,.F.,(4,3,3,3,3,3,3,3,3,3,3,3,3,3,3,3,
3,4),(0.,4.29652152148382E-5,8.44519107513973E-5,0.000123669830862666,0.000159788877355585,
0.000170558847912623,0.000181218775907163,0.000181960046452376,0.000214460062643276,
0.000244755726198279,0.000255838271868941,0.000258503253867575,0.000261084955178753,
0.000289370476647672,0.000301101325502006,0.000321109510663632,0.000331113603244445,
0.000341117695825258),.UNSPECIFIED.);
#4719=B_SPLINE_CURVE_WITH_KNOTS('',3,(#197176,#197177,#197178,#197179,#197180,
#197181,#197182,#197183,#197184,#197185,#197186,#197187,#197188,#197189,
#197190,#197191,#197192,#197193,#197194,#197195,#197196,#197197,#197198,
#197199,#197200,#197201,#197202,#197203,#197204,#197205,#197206,#197207,
#197208,#197209,#197210,#197211,#197212,#197213,#197214,#197215,#197216,
#197217,#197218,#197219,#197220,#197221,#197222,#197223,#197224,#197225,
#197226,#197227),.UNSPECIFIED.,.F.,.F.,(4,3,3,3,3,3,3,3,3,3,3,3,3,3,3,3,
3,4),(0.,4.30706237889783E-5,8.47417087733069E-5,0.000124159989210858,0.000160467076296833,
0.000170998382116681,0.000182414994733743,0.000213747977645858,0.000242415955903097,
0.000256497573175036,0.000259169422895609,0.000261757777312415,0.000289965130403247,
0.000301877270772902,0.000321937017503146,0.000326951954185707,0.000334474359209549,
0.00034199676423339),.UNSPECIFIED.);
#4720=B_SPLINE_CURVE_WITH_KNOTS('',3,(#197228,#197229,#197230,#197231,#197232,
#197233,#197234,#197235,#197236,#197237,#197238,#197239,#197240,#197241,
#197242,#197243,#197244,#197245,#197246,#197247,#197248,#197249,#197250,
#197251,#197252,#197253,#197254,#197255,#197256,#197257,#197258,#197259,
#197260,#197261,#197262,#197263,#197264,#197265,#197266,#197267,#197268,
#197269,#197270,#197271,#197272,#197273,#197274,#197275,#197276,#197277,
#197278,#197279),.UNSPECIFIED.,.F.,.F.,(4,3,3,3,3,3,3,3,3,3,3,3,3,3,3,3,
3,4),(3.46944695195361E-18,2.58457451679395E-5,4.25394446196648E-5,6.46659869687534E-5,
7.57292581432977E-5,8.12608937305698E-5,8.26438026273878E-5,8.67925293178419E-5,
0.000116015624428513,0.000130188793976761,0.000151886926306221,0.00016196365121127,
0.000162735992470951,0.00017358505863568,0.000212487880461813,0.000255238173513001,
0.000301397761148148,0.000347170117271353),.UNSPECIFIED.);
#4721=B_SPLINE_CURVE_WITH_KNOTS('',3,(#197281,#197282,#197283,#197284,#197285,
#197286,#197287,#197288,#197289,#197290,#197291,#197292,#197293,#197294,
#197295,#197296,#197297,#197298,#197299,#197300,#197301,#197302,#197303,
#197304,#197305,#197306,#197307,#197308,#197309,#197310,#197311,#197312,
#197313,#197314,#197315,#197316,#197317,#197318,#197319,#197320,#197321,
#197322,#197323,#197324,#197325,#197326),.UNSPECIFIED.,.F.,.F.,(4,3,3,3,
3,3,3,3,3,3,3,3,3,3,3,4),(0.,2.57218161995894E-5,4.21568322567858E-5,6.4587331461702E-5,
7.58025810641601E-5,8.14102058653892E-5,8.28121120656964E-5,8.70178306666182E-5,
0.000116081955658822,0.000130526745999927,0.000162394111022044,0.000174035661333236,
0.000213138396956959,0.000256116935431279,0.000302406662852392,0.000348071322666469),
 .UNSPECIFIED.);
#4722=B_SPLINE_CURVE_WITH_KNOTS('',3,(#197327,#197328,#197329,#197330,#197331,
#197332,#197333,#197334,#197335,#197336,#197337,#197338,#197339,#197340,
#197341,#197342,#197343,#197344,#197345,#197346,#197347,#197348,#197349,
#197350,#197351,#197352,#197353,#197354,#197355,#197356,#197357,#197358,
#197359,#197360,#197361,#197362,#197363,#197364,#197365,#197366,#197367,
#197368,#197369,#197370,#197371,#197372,#197373,#197374,#197375,#197376,
#197377,#197378),.UNSPECIFIED.,.F.,.F.,(4,3,3,3,3,3,3,3,3,3,3,3,3,3,3,3,
3,4),(0.,4.29652152094933E-5,8.44519107431452E-5,0.000123669830853246,0.000159788877346178,
0.000170558847912626,0.000181218775907166,0.000181960046452406,0.000214460062643372,
0.000244755726197706,0.000255838271868949,0.000258503253867584,0.000261084955178762,
0.000289370476648327,0.000301101325502017,0.000321109510663644,0.000331113603244458,
0.000341117695825272),.UNSPECIFIED.);
#4723=B_SPLINE_CURVE_WITH_KNOTS('',3,(#197380,#197381,#197382,#197383,#197384,
#197385,#197386,#197387,#197388,#197389,#197390,#197391,#197392,#197393,
#197394,#197395,#197396,#197397,#197398,#197399,#197400,#197401,#197402,
#197403,#197404,#197405,#197406,#197407,#197408,#197409,#197410,#197411,
#197412,#197413,#197414,#197415,#197416,#197417,#197418,#197419,#197420,
#197421,#197422,#197423,#197424,#197425,#197426,#197427,#197428,#197429,
#197430,#197431),.UNSPECIFIED.,.F.,.F.,(4,3,3,3,3,3,3,3,3,3,3,3,3,3,3,3,
3,4),(0.,4.30706237876313E-5,8.47417087707628E-5,0.000124159989207121,0.000160467076291592,
0.000170998382116703,0.00018241499473379,0.000213747977645873,0.000242415955903416,
0.000256497573175044,0.000259169422895617,0.000261757777312422,0.00028996513040352,
0.000301877270772903,0.000321937017503144,0.000326951954185704,0.000334474359209544,
0.000341996764233385),.UNSPECIFIED.);
#4724=B_SPLINE_CURVE_WITH_KNOTS('',3,(#197432,#197433,#197434,#197435,#197436,
#197437,#197438,#197439,#197440,#197441,#197442,#197443,#197444,#197445,
#197446,#197447,#197448,#197449,#197450,#197451,#197452,#197453,#197454,
#197455,#197456,#197457,#197458,#197459,#197460,#197461,#197462,#197463,
#197464,#197465,#197466,#197467,#197468,#197469,#197470,#197471,#197472,
#197473,#197474,#197475,#197476,#197477,#197478,#197479,#197480,#197481,
#197482,#197483),.UNSPECIFIED.,.F.,.F.,(4,3,3,3,3,3,3,3,3,3,3,3,3,3,3,3,
3,4),(0.,2.58457451665638E-5,4.25394446195485E-5,6.4665986968694E-5,7.57292581432668E-5,
8.12608937305532E-5,8.26438026273748E-5,8.67925293178396E-5,0.000116015624426654,
0.000130188793976759,0.000151886926306219,0.00016196365121128,0.000162735992470949,
0.000173585058635679,0.000212487880458713,0.00025523817350687,0.000301397761138754,
0.000347170117271368),.UNSPECIFIED.);
#4725=B_SPLINE_CURVE_WITH_KNOTS('',3,(#197485,#197486,#197487,#197488,#197489,
#197490,#197491,#197492,#197493,#197494,#197495,#197496,#197497,#197498,
#197499,#197500,#197501,#197502,#197503,#197504,#197505,#197506,#197507,
#197508,#197509,#197510,#197511,#197512,#197513,#197514,#197515,#197516,
#197517,#197518,#197519,#197520,#197521,#197522,#197523,#197524,#197525,
#197526,#197527,#197528,#197529,#197530),.UNSPECIFIED.,.F.,.F.,(4,3,3,3,
3,3,3,3,3,3,3,3,3,3,3,4),(0.,2.57218162017605E-5,4.21568322567747E-5,6.45873314616954E-5,
7.58025810641557E-5,8.14102058653859E-5,8.28121120656934E-5,8.7017830666616E-5,
0.000116081955659622,0.000130526745999924,0.000162394111022032,0.000174035661333232,
0.000213138396958048,0.000256116935433517,0.00030240666285608,0.000348071322666468),
 .UNSPECIFIED.);
#4726=B_SPLINE_CURVE_WITH_KNOTS('',3,(#197531,#197532,#197533,#197534,#197535,
#197536,#197537,#197538,#197539,#197540,#197541,#197542,#197543,#197544,
#197545,#197546,#197547,#197548,#197549,#197550,#197551,#197552,#197553,
#197554,#197555,#197556,#197557,#197558,#197559,#197560,#197561,#197562,
#197563,#197564,#197565,#197566,#197567,#197568,#197569,#197570,#197571,
#197572,#197573,#197574,#197575,#197576,#197577,#197578,#197579,#197580,
#197581,#197582),.UNSPECIFIED.,.F.,.F.,(4,3,3,3,3,3,3,3,3,3,3,3,3,3,3,3,
3,4),(0.,4.29652152129689E-5,8.44519107480275E-5,0.000123669830857744,0.000159788877348903,
0.000170558847912613,0.000181218775907154,0.000181960046452395,0.000214460062643831,
0.000244755726199015,0.000255838271868934,0.000258503253867569,0.000261084955178747,
0.000289370476647275,0.000301101325502001,0.000321109510663628,0.000331113603244442,
0.000341117695825255),.UNSPECIFIED.);
#4727=B_SPLINE_CURVE_WITH_KNOTS('',3,(#197584,#197585,#197586,#197587,#197588,
#197589,#197590,#197591,#197592,#197593,#197594,#197595,#197596,#197597,
#197598,#197599,#197600,#197601,#197602,#197603,#197604,#197605,#197606,
#197607,#197608,#197609,#197610,#197611,#197612,#197613,#197614,#197615,
#197616,#197617,#197618,#197619,#197620,#197621,#197622,#197623,#197624,
#197625,#197626,#197627,#197628,#197629,#197630,#197631,#197632,#197633,
#197634,#197635),.UNSPECIFIED.,.F.,.F.,(4,3,3,3,3,3,3,3,3,3,3,3,3,3,3,3,
3,4),(1.04083408558608E-17,4.307062378596E-5,8.47417087679539E-5,0.000124159989203457,
0.000160467076287138,0.000170998382116702,0.000182414994733776,0.000213747977645871,
0.000242415955902389,0.000256497573175041,0.000259169422895614,0.000261757777312419,
0.000289965130404368,0.000301877270772899,0.000321937017503139,0.000326951954185699,
0.00033447435920954,0.00034199676423338),.UNSPECIFIED.);
#4728=B_SPLINE_CURVE_WITH_KNOTS('',3,(#197636,#197637,#197638,#197639,#197640,
#197641,#197642,#197643,#197644,#197645,#197646,#197647,#197648,#197649,
#197650,#197651,#197652,#197653,#197654,#197655,#197656,#197657,#197658,
#197659,#197660,#197661,#197662,#197663,#197664,#197665,#197666,#197667,
#197668,#197669,#197670,#197671,#197672,#197673,#197674,#197675,#197676,
#197677,#197678,#197679,#197680,#197681,#197682,#197683,#197684,#197685,
#197686,#197687),.UNSPECIFIED.,.F.,.F.,(4,3,3,3,3,3,3,3,3,3,3,3,3,3,3,3,
3,4),(0.,2.58457451687787E-5,4.25394446196238E-5,6.46659869687319E-5,7.57292581432859E-5,
8.12608937305629E-5,8.26438026273822E-5,8.679252931784E-5,0.000116015624426979,
0.00013018879397676,0.00015188692630622,0.000161963651211278,0.00016273599247095,
0.00017358505863568,0.000212487880458027,0.000255238173505867,0.00030139776113807,
0.000347170117271346),.UNSPECIFIED.);
#4729=B_SPLINE_CURVE_WITH_KNOTS('',3,(#197689,#197690,#197691,#197692,#197693,
#197694,#197695,#197696,#197697,#197698,#197699,#197700,#197701,#197702,
#197703,#197704,#197705,#197706,#197707,#197708,#197709,#197710,#197711,
#197712,#197713,#197714,#197715,#197716,#197717,#197718,#197719,#197720,
#197721,#197722,#197723,#197724,#197725,#197726,#197727,#197728,#197729,
#197730,#197731,#197732,#197733,#197734),.UNSPECIFIED.,.F.,.F.,(4,3,3,3,
3,3,3,3,3,3,3,3,3,3,3,4),(0.,2.57218162007852E-5,4.21568322569827E-5,6.45873314618037E-5,
7.58025810642142E-5,8.14102058654194E-5,8.28121120657208E-5,8.70178306666247E-5,
0.000116081955658545,0.000130526745999937,0.000162394111022054,0.000174035661333249,
0.000213138396956967,0.00025611693543107,0.000302406662851331,0.000348071322666473),
 .UNSPECIFIED.);
#4730=B_SPLINE_CURVE_WITH_KNOTS('',3,(#197735,#197736,#197737,#197738,#197739,
#197740,#197741,#197742,#197743,#197744,#197745,#197746,#197747,#197748,
#197749,#197750,#197751,#197752,#197753,#197754,#197755,#197756,#197757,
#197758,#197759,#197760,#197761,#197762,#197763,#197764,#197765,#197766,
#197767,#197768,#197769,#197770,#197771,#197772,#197773,#197774,#197775,
#197776,#197777,#197778,#197779,#197780,#197781,#197782,#197783,#197784,
#197785,#197786),.UNSPECIFIED.,.F.,.F.,(4,3,3,3,3,3,3,3,3,3,3,3,3,3,3,3,
3,4),(0.,4.2965215213286E-5,8.44519107492582E-5,0.000123669830860511,0.000159788877354162,
0.000170558847912629,0.000181218775907169,0.000181960046452393,0.000214460062644021,
0.000244755726199397,0.00025583827186895,0.000258503253867585,0.000261084955178762,
0.000289370476647532,0.000301101325502016,0.000321109510663643,0.000331113603244457,
0.00034111769582527),.UNSPECIFIED.);
#4731=B_SPLINE_CURVE_WITH_KNOTS('',3,(#197788,#197789,#197790,#197791,#197792,
#197793,#197794,#197795,#197796,#197797,#197798,#197799,#197800,#197801,
#197802,#197803,#197804,#197805,#197806,#197807,#197808,#197809,#197810,
#197811,#197812,#197813,#197814,#197815,#197816,#197817,#197818,#197819,
#197820,#197821,#197822,#197823,#197824,#197825,#197826,#197827,#197828,
#197829,#197830,#197831,#197832,#197833,#197834,#197835,#197836,#197837,
#197838,#197839),.UNSPECIFIED.,.F.,.F.,(4,3,3,3,3,3,3,3,3,3,3,3,3,3,3,3,
3,4),(0.,4.30706237867224E-5,8.4741708769075E-5,0.000124159989204539,0.000160467076288079,
0.000170998382116707,0.000182414994733804,0.000213747977645877,0.000242415955904902,
0.000256497573175047,0.00025916942289562,0.000261757777312425,0.00028996513040259,
0.000301877270772906,0.000321937017503147,0.000326951954185707,0.000334474359209547,
0.000341996764233387),.UNSPECIFIED.);
#4732=B_SPLINE_CURVE_WITH_KNOTS('',3,(#197840,#197841,#197842,#197843,#197844,
#197845,#197846,#197847,#197848,#197849,#197850,#197851,#197852,#197853,
#197854,#197855,#197856,#197857,#197858,#197859,#197860,#197861,#197862,
#197863,#197864,#197865,#197866,#197867,#197868,#197869,#197870,#197871,
#197872,#197873,#197874,#197875,#197876,#197877,#197878,#197879,#197880,
#197881,#197882,#197883,#197884,#197885,#197886,#197887,#197888,#197889,
#197890,#197891),.UNSPECIFIED.,.F.,.F.,(4,3,3,3,3,3,3,3,3,3,3,3,3,3,3,3,
3,4),(0.,2.58457451687167E-5,4.25394446195716E-5,6.4665986968707E-5,7.57292581432747E-5,
8.12608937305585E-5,8.26438026273795E-5,8.67925293178424E-5,0.000116015624428119,
0.000130188793976764,0.000151886926306224,0.00016196365121127,0.000162735992470954,
0.000173585058635685,0.000212487880460168,0.000255238173509542,0.000301397761142473,
0.000347170117271368),.UNSPECIFIED.);
#4733=B_SPLINE_CURVE_WITH_KNOTS('',3,(#197893,#197894,#197895,#197896,#197897,
#197898,#197899,#197900,#197901,#197902,#197903,#197904,#197905,#197906,
#197907,#197908,#197909,#197910,#197911,#197912,#197913,#197914,#197915,
#197916,#197917,#197918,#197919,#197920,#197921,#197922,#197923,#197924,
#197925,#197926,#197927,#197928,#197929,#197930,#197931,#197932,#197933,
#197934,#197935,#197936,#197937,#197938),.UNSPECIFIED.,.F.,.F.,(4,3,3,3,
3,3,3,3,3,3,3,3,3,3,3,4),(0.,2.57218161993116E-5,4.21568322567207E-5,6.458733146167E-5,
7.58025810641446E-5,8.14102058653819E-5,8.28121120656913E-5,8.70178306666193E-5,
0.000116081955658386,0.000130526745999929,0.000162394111022047,0.000174035661333239,
0.000213138396957292,0.000256116935431947,0.00030240666285341,0.000348071322666464),
 .UNSPECIFIED.);
#4734=B_SPLINE_CURVE_WITH_KNOTS('',3,(#197939,#197940,#197941,#197942,#197943,
#197944,#197945,#197946,#197947,#197948,#197949,#197950,#197951,#197952,
#197953,#197954,#197955,#197956,#197957,#197958,#197959,#197960,#197961,
#197962,#197963,#197964,#197965,#197966,#197967,#197968,#197969,#197970,
#197971,#197972,#197973,#197974,#197975,#197976,#197977,#197978,#197979,
#197980,#197981,#197982,#197983,#197984,#197985,#197986,#197987,#197988,
#197989,#197990),.UNSPECIFIED.,.F.,.F.,(4,3,3,3,3,3,3,3,3,3,3,3,3,3,3,3,
3,4),(0.,4.29652152170491E-5,8.44519107548311E-5,0.000123669830866424,0.000159788877359245,
0.000170558847912628,0.000181218775907168,0.000181960046452396,0.000214460062643474,
0.000244755726198156,0.000255838271868947,0.000258503253867582,0.00026108495517876,
0.000289370476647647,0.000301101325502013,0.00032110951066364,0.000331113603244453,
0.000341117695825266),.UNSPECIFIED.);
#4735=B_SPLINE_CURVE_WITH_KNOTS('',3,(#210566,#210567,#210568,#210569,#210570,
#210571,#210572,#210573,#210574,#210575,#210576,#210577,#210578,#210579,
#210580,#210581,#210582,#210583,#210584,#210585,#210586,#210587,#210588,
#210589,#210590,#210591,#210592,#210593,#210594,#210595,#210596,#210597,
#210598,#210599,#210600,#210601,#210602,#210603,#210604,#210605,#210606,
#210607,#210608),.UNSPECIFIED.,.F.,.F.,(4,3,3,3,3,3,3,3,3,3,3,3,3,3,4),
(1.00966327312713E-18,1.12890698065814E-5,7.65259667132928E-5,0.000102837507928491,
0.000112544869199234,0.000130746171581876,0.000194450729921123,0.000226303009090746,
0.000242229148675558,0.00025815528826037,0.000258291104876521,0.000327654633610499,
0.000399363990827472,0.000469709285179123,0.000516310576520739),
 .UNSPECIFIED.);
#4736=B_SPLINE_CURVE_WITH_KNOTS('',3,(#210616,#210617,#210618,#210619,#210620,
#210621,#210622,#210623,#210624,#210625,#210626,#210627,#210628,#210629,
#210630,#210631,#210632,#210633,#210634,#210635,#210636,#210637,#210638,
#210639,#210640,#210641,#210642,#210643,#210644,#210645,#210646,#210647,
#210648,#210649,#210650,#210651,#210652,#210653,#210654,#210655),
 .UNSPECIFIED.,.F.,.F.,(4,3,3,3,3,3,3,3,3,3,3,3,3,4),(4.33680868994202E-19,
6.84564250796869E-5,0.000138288406590208,0.000205407478923098,0.000256966021225852,
0.000257101146970264,0.000271589374668167,0.000352213067611634,0.000388398097499792,
0.000404123622054884,0.000459162957997706,0.000486682625969117,0.000500442459954822,
0.000514202293940528),.UNSPECIFIED.);
#4737=B_SPLINE_CURVE_WITH_KNOTS('',3,(#210659,#210660,#210661,#210662,#210663,
#210664,#210665,#210666,#210667,#210668,#210669,#210670,#210671,#210672,
#210673,#210674,#210675,#210676,#210677,#210678,#210679,#210680,#210681,
#210682,#210683,#210684,#210685,#210686,#210687,#210688,#210689,#210690,
#210691,#210692,#210693,#210694,#210695,#210696,#210697,#210698,#210699,
#210700,#210701),.UNSPECIFIED.,.F.,.F.,(4,3,3,3,3,3,3,3,3,3,3,3,3,3,4),
(8.67361737988403E-19,1.12890698065815E-5,7.65259667117838E-5,0.000102837507928496,
0.000112544869199238,0.00013074617158188,0.000194450729921126,0.000226303009090749,
0.000242229148675561,0.000258155288260372,0.000258291104876519,0.000327654633617137,
0.000399363990840869,0.000469709285198284,0.000516310576520743),
 .UNSPECIFIED.);
#4738=B_SPLINE_CURVE_WITH_KNOTS('',3,(#210709,#210710,#210711,#210712,#210713,
#210714,#210715,#210716,#210717,#210718,#210719,#210720,#210721,#210722,
#210723,#210724,#210725,#210726,#210727,#210728,#210729,#210730,#210731,
#210732,#210733,#210734,#210735,#210736,#210737,#210738,#210739,#210740,
#210741,#210742,#210743,#210744,#210745,#210746,#210747,#210748),
 .UNSPECIFIED.,.F.,.F.,(4,3,3,3,3,3,3,3,3,3,3,3,3,4),(4.33680868994202E-19,
6.84564250822044E-5,0.000138288406595129,0.000205407478930009,0.000256966021225841,
0.000257101146970262,0.000271589374668164,0.000352213067605997,0.000388398097499794,
0.000404123622054885,0.000459162957997704,0.000486682625969113,0.000500442459954818,
0.000514202293940523),.UNSPECIFIED.);
#4739=B_SPLINE_CURVE_WITH_KNOTS('',3,(#210752,#210753,#210754,#210755,#210756,
#210757,#210758,#210759,#210760,#210761,#210762,#210763,#210764,#210765,
#210766,#210767,#210768,#210769,#210770,#210771,#210772,#210773,#210774,
#210775,#210776,#210777,#210778,#210779,#210780,#210781,#210782,#210783,
#210784,#210785,#210786,#210787,#210788,#210789,#210790,#210791,#210792,
#210793,#210794),.UNSPECIFIED.,.F.,.F.,(4,3,3,3,3,3,3,3,3,3,3,3,3,3,4),
(1.73472347597681E-18,1.12890698065814E-5,7.65259667015125E-5,0.000102837507928481,
0.000112544869199225,0.000130746171581868,0.000194450729921122,0.000226303009090748,
0.000242229148675561,0.000258155288260375,0.000258291104876516,0.000327654633617638,
0.000399363990841712,0.000469709285199623,0.000516310576520747),
 .UNSPECIFIED.);
#4740=B_SPLINE_CURVE_WITH_KNOTS('',3,(#210802,#210803,#210804,#210805,#210806,
#210807,#210808,#210809,#210810,#210811,#210812,#210813,#210814,#210815,
#210816,#210817,#210818,#210819,#210820,#210821,#210822,#210823,#210824,
#210825,#210826,#210827,#210828,#210829,#210830,#210831,#210832,#210833,
#210834,#210835,#210836,#210837,#210838,#210839,#210840,#210841),
 .UNSPECIFIED.,.F.,.F.,(4,3,3,3,3,3,3,3,3,3,3,3,3,4),(8.67361737988404E-19,
6.84564250848222E-5,0.000138288406600658,0.000205407478938653,0.000256966021225847,
0.00025710114697026,0.000271589374668165,0.00035221306760003,0.000388398097499774,
0.000404123622054867,0.000459162957997694,0.000486682625969107,0.000500442459954813,
0.00051420229394052),.UNSPECIFIED.);
#4741=B_SPLINE_CURVE_WITH_KNOTS('',3,(#210845,#210846,#210847,#210848,#210849,
#210850,#210851,#210852,#210853,#210854,#210855,#210856,#210857,#210858,
#210859,#210860,#210861,#210862,#210863,#210864,#210865,#210866,#210867,
#210868,#210869,#210870,#210871,#210872,#210873,#210874,#210875,#210876,
#210877,#210878,#210879,#210880,#210881,#210882,#210883,#210884,#210885,
#210886,#210887),.UNSPECIFIED.,.F.,.F.,(4,3,3,3,3,3,3,3,3,3,3,3,3,3,4),
(0.,1.12890698065831E-5,7.65259667075185E-5,0.000102837507928526,0.000112544869199266,
0.000130746171581904,0.000194450729921138,0.000226303009090756,0.000242229148675564,
0.000258155288260373,0.0002582911048765,0.000327654633616213,0.000399363990838748,
0.000469709285194883,0.000516310576520745),.UNSPECIFIED.);
#4742=B_SPLINE_CURVE_WITH_KNOTS('',3,(#210895,#210896,#210897,#210898,#210899,
#210900,#210901,#210902,#210903,#210904,#210905,#210906,#210907,#210908,
#210909,#210910,#210911,#210912,#210913,#210914,#210915,#210916,#210917,
#210918,#210919,#210920,#210921,#210922,#210923,#210924,#210925,#210926,
#210927,#210928,#210929,#210930,#210931,#210932,#210933,#210934),
 .UNSPECIFIED.,.F.,.F.,(4,3,3,3,3,3,3,3,3,3,3,3,3,4),(1.30104260698261E-18,
6.84564250769938E-5,0.000138288406585387,0.000205407478917741,0.000256966021225848,
0.000257101146970264,0.000271589374668167,0.000352213067597738,0.000388398097499812,
0.000404123622054901,0.000459162957997714,0.000486682625969121,0.000500442459954824,
0.000514202293940527),.UNSPECIFIED.);
#4743=B_SPLINE_CURVE_WITH_KNOTS('',3,(#210938,#210939,#210940,#210941,#210942,
#210943,#210944,#210945,#210946,#210947,#210948,#210949,#210950,#210951,
#210952,#210953,#210954,#210955,#210956,#210957,#210958,#210959,#210960,
#210961,#210962,#210963,#210964,#210965,#210966,#210967,#210968,#210969,
#210970,#210971,#210972,#210973,#210974,#210975,#210976,#210977,#210978,
#210979,#210980),.UNSPECIFIED.,.F.,.F.,(4,3,3,3,3,3,3,3,3,3,3,3,3,3,4),
(3.49644694633735E-18,1.12890698065849E-5,7.65259667044717E-5,0.000102837507928498,
0.00011254486919924,0.000130746171581882,0.00019445072992113,0.000226303009090754,
0.000242229148675566,0.000258155288260378,0.000258291104876529,0.000327654633621337,
0.000399363990849304,0.000469709285210601,0.000516310576520752),
 .UNSPECIFIED.);
#4744=B_SPLINE_CURVE_WITH_KNOTS('',3,(#210988,#210989,#210990,#210991,#210992,
#210993,#210994,#210995,#210996,#210997,#210998,#210999,#211000,#211001,
#211002,#211003,#211004,#211005,#211006,#211007,#211008,#211009,#211010,
#211011,#211012,#211013,#211014,#211015,#211016,#211017,#211018,#211019,
#211020,#211021,#211022,#211023,#211024,#211025,#211026,#211027),
 .UNSPECIFIED.,.F.,.F.,(4,3,3,3,3,3,3,3,3,3,3,3,3,4),(1.30104260698261E-18,
6.84564250824312E-5,0.000138288406595942,0.000205407478931792,0.000256966021225845,
0.000257101146970262,0.00027158937466816,0.000352213067614797,0.000388398097499752,
0.000404123622054848,0.000459162957997682,0.000486682625969099,0.000500442459954807,
0.000514202293940516),.UNSPECIFIED.);
#4745=B_SPLINE_CURVE_WITH_KNOTS('',3,(#211031,#211032,#211033,#211034,#211035,
#211036,#211037,#211038,#211039,#211040,#211041,#211042,#211043,#211044,
#211045,#211046,#211047,#211048,#211049,#211050,#211051,#211052,#211053,
#211054,#211055,#211056,#211057,#211058,#211059,#211060,#211061,#211062,
#211063,#211064,#211065,#211066,#211067,#211068,#211069,#211070,#211071,
#211072,#211073),.UNSPECIFIED.,.F.,.F.,(4,3,3,3,3,3,3,3,3,3,3,3,3,3,4),
(0.,1.12890698065827E-5,7.65259667060974E-5,0.00010283750792849,0.000112544869199233,
0.000130746171581877,0.000194450729921129,0.000226303009090755,0.000242229148675568,
0.000258155288260381,0.000258291104876531,0.000327654633612254,0.000399363990830589,
0.000469709285182946,0.000516310576520763),.UNSPECIFIED.);
#4746=B_SPLINE_CURVE_WITH_KNOTS('',3,(#211081,#211082,#211083,#211084,#211085,
#211086,#211087,#211088,#211089,#211090,#211091,#211092,#211093,#211094,
#211095,#211096,#211097,#211098,#211099,#211100,#211101,#211102,#211103,
#211104,#211105,#211106,#211107,#211108,#211109,#211110,#211111,#211112,
#211113,#211114,#211115,#211116,#211117,#211118,#211119,#211120),
 .UNSPECIFIED.,.F.,.F.,(4,3,3,3,3,3,3,3,3,3,3,3,3,4),(2.60208521396521E-18,
6.84564250839596E-5,0.000138288406599065,0.00020540747893661,0.000256966021225842,
0.000257101146970262,0.000271589374668167,0.000352213067605811,0.000388398097499827,
0.000404123622054914,0.000459162957997718,0.00048668262596912,0.000500442459954821,
0.000514202293940522),.UNSPECIFIED.);
#4747=B_SPLINE_CURVE_WITH_KNOTS('',3,(#211124,#211125,#211126,#211127,#211128,
#211129,#211130,#211131,#211132,#211133,#211134,#211135,#211136,#211137,
#211138,#211139,#211140,#211141,#211142,#211143,#211144,#211145,#211146,
#211147,#211148,#211149,#211150,#211151,#211152,#211153,#211154,#211155,
#211156,#211157,#211158,#211159,#211160,#211161,#211162,#211163,#211164,
#211165,#211166),.UNSPECIFIED.,.F.,.F.,(4,3,3,3,3,3,3,3,3,3,3,3,3,3,4),
(0.,1.12890698065808E-5,7.65259667096804E-5,0.00010283750792849,0.000112544869199233,
0.000130746171581876,0.000194450729921126,0.000226303009090751,0.000242229148675564,
0.000258155288260376,0.000258291104876522,0.00032765463361035,0.000399363990827097,
0.000469709285178512,0.000516310576520752),.UNSPECIFIED.);
#4748=B_SPLINE_CURVE_WITH_KNOTS('',3,(#211174,#211175,#211176,#211177,#211178,
#211179,#211180,#211181,#211182,#211183,#211184,#211185,#211186,#211187,
#211188,#211189,#211190,#211191,#211192,#211193,#211194,#211195,#211196,
#211197,#211198,#211199,#211200,#211201,#211202,#211203,#211204,#211205,
#211206,#211207,#211208,#211209,#211210,#211211,#211212,#211213),
 .UNSPECIFIED.,.F.,.F.,(4,3,3,3,3,3,3,3,3,3,3,3,3,4),(0.,6.84564250845964E-5,
0.00013828840659994,0.000205407478937272,0.000256966021225841,0.000257101146970266,
0.000271589374668168,0.000352213067593158,0.000388398097499835,0.000404123622054922,
0.000459162957997727,0.00048668262596913,0.000500442459954831,0.000514202293940532),
 .UNSPECIFIED.);
#4749=B_SPLINE_CURVE_WITH_KNOTS('',3,(#211217,#211218,#211219,#211220,#211221,
#211222,#211223,#211224,#211225,#211226,#211227,#211228,#211229,#211230,
#211231,#211232,#211233,#211234,#211235,#211236,#211237,#211238,#211239,
#211240,#211241,#211242,#211243,#211244,#211245,#211246,#211247,#211248,
#211249,#211250,#211251,#211252,#211253,#211254,#211255,#211256,#211257,
#211258,#211259),.UNSPECIFIED.,.F.,.F.,(4,3,3,3,3,3,3,3,3,3,3,3,3,3,4),
(0.,1.12890698065865E-5,7.65259667038362E-5,0.000102837507928542,0.000112544869199282,
0.00013074617158192,0.00019445072992115,0.000226303009090765,0.000242229148675573,
0.000258155288260381,0.00025829110487653,0.000327654633624173,0.000399363990855843,
0.000469709285221651,0.000516310576520761),.UNSPECIFIED.);
#4750=B_SPLINE_CURVE_WITH_KNOTS('',3,(#211267,#211268,#211269,#211270,#211271,
#211272,#211273,#211274,#211275,#211276,#211277,#211278,#211279,#211280,
#211281,#211282,#211283,#211284,#211285,#211286,#211287,#211288,#211289,
#211290,#211291,#211292,#211293,#211294,#211295,#211296,#211297,#211298,
#211299,#211300,#211301,#211302,#211303,#211304,#211305,#211306),
 .UNSPECIFIED.,.F.,.F.,(4,3,3,3,3,3,3,3,3,3,3,3,3,4),(0.,6.84564250818784E-5,
0.000138288406593889,0.000205407478926654,0.000256966021225852,0.000257101146970261,
0.000271589374668155,0.000352213067609107,0.000388398097499764,0.000404123622054859,
0.000459162957997691,0.000486682625969106,0.000500442459954814,0.000514202293940522),
 .UNSPECIFIED.);
#4751=B_SPLINE_CURVE_WITH_KNOTS('',3,(#211310,#211311,#211312,#211313,#211314,
#211315,#211316,#211317,#211318,#211319,#211320,#211321,#211322,#211323,
#211324,#211325,#211326,#211327,#211328,#211329,#211330,#211331,#211332,
#211333,#211334,#211335,#211336,#211337,#211338,#211339,#211340,#211341,
#211342,#211343,#211344,#211345,#211346,#211347,#211348,#211349,#211350,
#211351,#211352),.UNSPECIFIED.,.F.,.F.,(4,3,3,3,3,3,3,3,3,3,3,3,3,3,4),
(0.,1.12890698065827E-5,7.65259666926421E-5,0.00010283750792851,0.000112544869199251,
0.000130746171581891,0.00019445072992113,0.00022630300909075,0.00024222914867556,
0.00025815528826037,0.000258291104876511,0.000327654633619911,0.000399363990845548,
0.000469709285203805,0.00051631057652074),.UNSPECIFIED.);
#4752=B_SPLINE_CURVE_WITH_KNOTS('',3,(#211360,#211361,#211362,#211363,#211364,
#211365,#211366,#211367,#211368,#211369,#211370,#211371,#211372,#211373,
#211374,#211375,#211376,#211377,#211378,#211379,#211380,#211381,#211382,
#211383,#211384,#211385,#211386,#211387,#211388,#211389,#211390,#211391,
#211392,#211393,#211394,#211395,#211396,#211397,#211398,#211399),
 .UNSPECIFIED.,.F.,.F.,(4,3,3,3,3,3,3,3,3,3,3,3,3,4),(0.,6.84564250825335E-5,
0.000138288406596393,0.000205407478932587,0.000256966021225845,0.000257101146970255,
0.000271589374668162,0.00035221306762113,0.00038839809749983,0.000404123622054915,
0.000459162957997712,0.000486682625969111,0.00050044245995481,0.000514202293940509),
 .UNSPECIFIED.);
#4753=B_SPLINE_CURVE_WITH_KNOTS('',3,(#211403,#211404,#211405,#211406,#211407,
#211408,#211409,#211410,#211411,#211412,#211413,#211414,#211415,#211416,
#211417,#211418,#211419,#211420,#211421,#211422,#211423,#211424,#211425,
#211426,#211427,#211428,#211429,#211430,#211431,#211432,#211433,#211434,
#211435,#211436,#211437,#211438,#211439,#211440,#211441,#211442,#211443,
#211444,#211445),.UNSPECIFIED.,.F.,.F.,(4,3,3,3,3,3,3,3,3,3,3,3,3,3,4),
(0.,1.12890698065864E-5,7.65259667099654E-5,0.000102837507928553,0.000112544869199291,
0.000130746171581926,0.000194450729921147,0.000226303009090758,0.000242229148675563,
0.000258155288260369,0.000258291104876501,0.000327654633610913,0.000399363990828535,
0.000469709285181062,0.000516310576520738),.UNSPECIFIED.);
#4754=B_SPLINE_CURVE_WITH_KNOTS('',3,(#211453,#211454,#211455,#211456,#211457,
#211458,#211459,#211460,#211461,#211462,#211463,#211464,#211465,#211466,
#211467,#211468,#211469,#211470,#211471,#211472,#211473,#211474,#211475,
#211476,#211477,#211478,#211479,#211480,#211481,#211482,#211483,#211484,
#211485,#211486,#211487,#211488,#211489,#211490,#211491,#211492),
 .UNSPECIFIED.,.F.,.F.,(4,3,3,3,3,3,3,3,3,3,3,3,3,4),(4.33680868994202E-19,
6.84564250886368E-5,0.000138288406607453,0.000205407478945846,0.000256966021225854,
0.000257101146970262,0.00027158937466817,0.000352213067613361,0.000388398097499844,
0.000404123622054929,0.000459162957997726,0.000486682625969125,0.000500442459954824,
0.000514202293940523),.UNSPECIFIED.);
#4755=B_SPLINE_CURVE_WITH_KNOTS('',3,(#211496,#211497,#211498,#211499,#211500,
#211501,#211502,#211503,#211504,#211505,#211506,#211507,#211508,#211509,
#211510,#211511,#211512,#211513,#211514,#211515,#211516,#211517,#211518,
#211519,#211520,#211521,#211522,#211523,#211524,#211525,#211526,#211527,
#211528,#211529,#211530,#211531,#211532,#211533,#211534,#211535,#211536,
#211537,#211538),.UNSPECIFIED.,.F.,.F.,(4,3,3,3,3,3,3,3,3,3,3,3,3,3,4),
(0.,1.12890698065847E-5,7.65259667058506E-5,0.000102837507928533,0.000112544869199273,
0.00013074617158191,0.000194450729921141,0.000226303009090757,0.000242229148675565,
0.000258155288260372,0.000258291104876516,0.000327654633608951,0.000399363990824417,
0.000469709285175076,0.000516310576520745),.UNSPECIFIED.);
#4756=B_SPLINE_CURVE_WITH_KNOTS('',3,(#211546,#211547,#211548,#211549,#211550,
#211551,#211552,#211553,#211554,#211555,#211556,#211557,#211558,#211559,
#211560,#211561,#211562,#211563,#211564,#211565,#211566,#211567,#211568,
#211569,#211570,#211571,#211572,#211573,#211574,#211575,#211576,#211577,
#211578,#211579,#211580,#211581,#211582,#211583,#211584,#211585),
 .UNSPECIFIED.,.F.,.F.,(4,3,3,3,3,3,3,3,3,3,3,3,3,4),(0.,6.84564250865644E-5,
0.000138288406603816,0.000205407478941927,0.000256966021225846,0.00025710114697026,
0.000271589374668163,0.000352213067623985,0.000388398097499785,0.000404123622054877,
0.000459162957997698,0.000486682625969109,0.000500442459954814,0.000514202293940519),
 .UNSPECIFIED.);
#4757=B_SPLINE_CURVE_WITH_KNOTS('',3,(#211589,#211590,#211591,#211592,#211593,
#211594,#211595,#211596,#211597,#211598,#211599,#211600,#211601,#211602,
#211603,#211604,#211605,#211606,#211607,#211608,#211609,#211610,#211611,
#211612,#211613,#211614,#211615,#211616,#211617,#211618,#211619,#211620,
#211621,#211622,#211623,#211624,#211625,#211626,#211627,#211628,#211629,
#211630,#211631),.UNSPECIFIED.,.F.,.F.,(4,3,3,3,3,3,3,3,3,3,3,3,3,3,4),
(0.,1.12890698065774E-5,7.65259667018237E-5,0.000102837507928468,0.000112544869199212,
0.000130746171581857,0.000194450729921116,0.000226303009090745,0.000242229148675559,
0.000258155288260374,0.000258291104876517,0.000327654633618882,0.000399363990844482,
0.000469709285204073,0.000516310576520747),.UNSPECIFIED.);
#4758=B_SPLINE_CURVE_WITH_KNOTS('',3,(#211639,#211640,#211641,#211642,#211643,
#211644,#211645,#211646,#211647,#211648,#211649,#211650,#211651,#211652,
#211653,#211654,#211655,#211656,#211657,#211658,#211659,#211660,#211661,
#211662,#211663,#211664,#211665,#211666,#211667,#211668,#211669,#211670,
#211671,#211672,#211673,#211674,#211675,#211676,#211677,#211678),
 .UNSPECIFIED.,.F.,.F.,(4,3,3,3,3,3,3,3,3,3,3,3,3,4),(0.,6.84564250816909E-5,
0.000138288406594364,0.000205407478929581,0.000256966021225844,0.000257101146970261,
0.000271589374668163,0.000352213067604973,0.000388398097499789,0.000404123622054881,
0.000459162957997701,0.000486682625969112,0.000500442459954817,0.000514202293940522),
 .UNSPECIFIED.);
#4759=B_SPLINE_CURVE_WITH_KNOTS('',3,(#211682,#211683,#211684,#211685,#211686,
#211687,#211688,#211689,#211690,#211691,#211692,#211693,#211694,#211695,
#211696,#211697,#211698,#211699,#211700,#211701,#211702,#211703,#211704,
#211705,#211706,#211707,#211708,#211709,#211710,#211711,#211712,#211713,
#211714,#211715,#211716,#211717,#211718,#211719,#211720,#211721,#211722,
#211723,#211724),.UNSPECIFIED.,.F.,.F.,(4,3,3,3,3,3,3,3,3,3,3,3,3,3,4),
(3.49644694633735E-18,1.12890698065813E-5,7.65259667019077E-5,0.000102837507928475,
0.000112544869199218,0.000130746171581863,0.000194450729921118,0.000226303009090746,
0.00024222914867556,0.000258155288260374,0.000258291104876514,0.00032765463360937,
0.000399363990824599,0.000469709285174166,0.000516310576520744),
 .UNSPECIFIED.);
#4760=B_SPLINE_CURVE_WITH_KNOTS('',3,(#211732,#211733,#211734,#211735,#211736,
#211737,#211738,#211739,#211740,#211741,#211742,#211743,#211744,#211745,
#211746,#211747,#211748,#211749,#211750,#211751,#211752,#211753,#211754,
#211755,#211756,#211757,#211758,#211759,#211760,#211761,#211762,#211763,
#211764,#211765,#211766,#211767,#211768,#211769,#211770,#211771),
 .UNSPECIFIED.,.F.,.F.,(4,3,3,3,3,3,3,3,3,3,3,3,3,4),(0.,6.84564250813522E-5,
0.00013828840659376,0.000205407478929029,0.000256966021225855,0.000257101146970262,
0.000271589374668161,0.000352213067597481,0.000388398097499751,0.000404123622054848,
0.000459162957997686,0.000486682625969105,0.000500442459954814,0.000514202293940524),
 .UNSPECIFIED.);
#4761=B_SPLINE_CURVE_WITH_KNOTS('',3,(#211775,#211776,#211777,#211778,#211779,
#211780,#211781,#211782,#211783,#211784,#211785,#211786,#211787,#211788,
#211789,#211790,#211791,#211792,#211793,#211794,#211795,#211796,#211797,
#211798,#211799,#211800,#211801,#211802,#211803,#211804,#211805,#211806,
#211807,#211808,#211809,#211810,#211811,#211812,#211813,#211814,#211815,
#211816,#211817),.UNSPECIFIED.,.F.,.F.,(4,3,3,3,3,3,3,3,3,3,3,3,3,3,4),
(1.73472347597681E-18,1.12890698065837E-5,7.65259667051301E-5,0.000102837507928518,
0.000112544869199259,0.000130746171581897,0.000194450729921133,0.000226303009090751,
0.00024222914867556,0.000258155288260369,0.000258291104876513,0.000327654633617816,
0.000399363990842313,0.000469709285200686,0.000516310576520726),
 .UNSPECIFIED.);
#4762=B_SPLINE_CURVE_WITH_KNOTS('',3,(#211825,#211826,#211827,#211828,#211829,
#211830,#211831,#211832,#211833,#211834,#211835,#211836,#211837,#211838,
#211839,#211840,#211841,#211842,#211843,#211844,#211845,#211846,#211847,
#211848,#211849,#211850,#211851,#211852,#211853,#211854,#211855,#211856,
#211857,#211858,#211859,#211860,#211861,#211862,#211863,#211864),
 .UNSPECIFIED.,.F.,.F.,(4,3,3,3,3,3,3,3,3,3,3,3,3,4),(0.,6.84564250894095E-5,
0.000138288406610231,0.000205407478953372,0.000256966021225845,0.000257101146970263,
0.000271589374668162,0.000352213067603236,0.000388398097499751,0.000404123622054848,
0.000459162957997687,0.000486682625969107,0.000500442459954817,0.000514202293940527),
 .UNSPECIFIED.);
#4763=B_SPLINE_CURVE_WITH_KNOTS('',3,(#211868,#211869,#211870,#211871,#211872,
#211873,#211874,#211875,#211876,#211877,#211878,#211879,#211880,#211881,
#211882,#211883,#211884,#211885,#211886,#211887,#211888,#211889,#211890,
#211891,#211892,#211893,#211894,#211895,#211896,#211897,#211898,#211899,
#211900,#211901,#211902,#211903,#211904,#211905,#211906,#211907,#211908,
#211909,#211910),.UNSPECIFIED.,.F.,.F.,(4,3,3,3,3,3,3,3,3,3,3,3,3,3,4),
(0.,1.12890698065877E-5,7.65259667073395E-5,0.000102837507928553,0.000112544869199292,
0.000130746171581928,0.000194450729921153,0.000226303009090765,0.000242229148675571,
0.000258155288260377,0.000258291104876526,0.000327654633615,0.00039936399083635,
0.000469709285191737,0.000516310576520754),.UNSPECIFIED.);
#4764=B_SPLINE_CURVE_WITH_KNOTS('',3,(#211918,#211919,#211920,#211921,#211922,
#211923,#211924,#211925,#211926,#211927,#211928,#211929,#211930,#211931,
#211932,#211933,#211934,#211935,#211936,#211937,#211938,#211939,#211940,
#211941,#211942,#211943,#211944,#211945,#211946,#211947,#211948,#211949,
#211950,#211951,#211952,#211953,#211954,#211955,#211956,#211957),
 .UNSPECIFIED.,.F.,.F.,(4,3,3,3,3,3,3,3,3,3,3,3,3,4),(0.,6.84564250787773E-5,
0.000138288406588452,0.000205407478920936,0.000256966021225854,0.000257101146970262,
0.000271589374668165,0.000352213067598457,0.000388398097499807,0.000404123622054896,
0.00045916295799771,0.000486682625969117,0.00050044245995482,0.000514202293940524),
 .UNSPECIFIED.);
#4765=B_SPLINE_CURVE_WITH_KNOTS('',3,(#211961,#211962,#211963,#211964,#211965,
#211966,#211967,#211968,#211969,#211970,#211971,#211972,#211973,#211974,
#211975,#211976,#211977,#211978,#211979,#211980,#211981,#211982,#211983,
#211984,#211985,#211986,#211987,#211988,#211989,#211990,#211991,#211992,
#211993,#211994,#211995,#211996,#211997,#211998,#211999,#212000,#212001,
#212002,#212003),.UNSPECIFIED.,.F.,.F.,(4,3,3,3,3,3,3,3,3,3,3,3,3,3,4),
(0.,1.12890698065883E-5,7.65259667085461E-5,0.00010283750792858,0.000112544869199317,
0.000130746171581948,0.000194450729921159,0.000226303009090765,0.000242229148675568,
0.00025815528826037,0.000258291104876529,0.000327654633609379,0.000399363990825211,
0.000469709285175903,0.000516310576520741),.UNSPECIFIED.);
#4766=B_SPLINE_CURVE_WITH_KNOTS('',3,(#212011,#212012,#212013,#212014,#212015,
#212016,#212017,#212018,#212019,#212020,#212021,#212022,#212023,#212024,
#212025,#212026,#212027,#212028,#212029,#212030,#212031,#212032,#212033,
#212034,#212035,#212036,#212037,#212038,#212039,#212040,#212041,#212042,
#212043,#212044,#212045,#212046,#212047,#212048,#212049,#212050),
 .UNSPECIFIED.,.F.,.F.,(4,3,3,3,3,3,3,3,3,3,3,3,3,4),(0.,6.84564250867182E-5,
0.000138288406604464,0.000205407478943975,0.000256966021225847,0.000257101146970263,
0.000271589374668164,0.000352213067606211,0.000388398097499806,0.000404123622054896,
0.000459162957997711,0.000486682625969118,0.000500442459954822,0.000514202293940525),
 .UNSPECIFIED.);
#4767=B_SPLINE_CURVE_WITH_KNOTS('',3,(#212054,#212055,#212056,#212057,#212058,
#212059,#212060,#212061,#212062,#212063,#212064,#212065,#212066,#212067,
#212068,#212069,#212070,#212071,#212072,#212073,#212074,#212075,#212076,
#212077,#212078,#212079,#212080,#212081,#212082,#212083,#212084,#212085,
#212086,#212087,#212088,#212089,#212090,#212091,#212092,#212093,#212094,
#212095,#212096),.UNSPECIFIED.,.F.,.F.,(4,3,3,3,3,3,3,3,3,3,3,3,3,3,4),
(8.67361737988404E-19,1.12890698065864E-5,7.65259667038092E-5,0.000102837507928523,
0.000112544869199264,0.000130746171581903,0.000194450729921138,0.000226303009090756,
0.000242229148675565,0.000258155288260374,0.000258291104876511,0.000327654633611257,
0.000399363990828871,0.000469709285181089,0.000516310576520747),
 .UNSPECIFIED.);
#4768=B_SPLINE_CURVE_WITH_KNOTS('',3,(#212104,#212105,#212106,#212107,#212108,
#212109,#212110,#212111,#212112,#212113,#212114,#212115,#212116,#212117,
#212118,#212119,#212120,#212121,#212122,#212123,#212124,#212125,#212126,
#212127,#212128,#212129,#212130,#212131,#212132,#212133,#212134,#212135,
#212136,#212137,#212138,#212139,#212140,#212141,#212142,#212143),
 .UNSPECIFIED.,.F.,.F.,(4,3,3,3,3,3,3,3,3,3,3,3,3,4),(4.33680868994202E-19,
6.84564250888431E-5,0.000138288406609379,0.000205407478952497,0.000256966021225853,
0.000257101146970263,0.000271589374668164,0.000352213067610745,0.000388398097499789,
0.000404123622054881,0.000459162957997703,0.000486682625969114,0.00050044245995482,
0.000514202293940525),.UNSPECIFIED.);
#4769=B_SPLINE_CURVE_WITH_KNOTS('',3,(#212147,#212148,#212149,#212150,#212151,
#212152,#212153,#212154,#212155,#212156,#212157,#212158,#212159,#212160,
#212161,#212162,#212163,#212164,#212165,#212166,#212167,#212168,#212169,
#212170,#212171,#212172,#212173,#212174,#212175,#212176,#212177,#212178,
#212179,#212180,#212181,#212182,#212183,#212184,#212185,#212186,#212187,
#212188,#212189),.UNSPECIFIED.,.F.,.F.,(4,3,3,3,3,3,3,3,3,3,3,3,3,3,4),
(1.73472347597681E-18,1.12890698065875E-5,7.65259667031789E-5,0.000102837507928535,
0.000112544869199274,0.000130746171581911,0.000194450729921138,0.000226303009090752,
0.000242229148675558,0.000258155288260365,0.000258291104876515,0.000327654633613017,
0.000399363990832523,0.000469709285186505,0.000516310576520729),
 .UNSPECIFIED.);
#4770=B_SPLINE_CURVE_WITH_KNOTS('',3,(#212197,#212198,#212199,#212200,#212201,
#212202,#212203,#212204,#212205,#212206,#212207,#212208,#212209,#212210,
#212211,#212212,#212213,#212214,#212215,#212216,#212217,#212218,#212219,
#212220,#212221,#212222,#212223,#212224,#212225,#212226,#212227,#212228,
#212229,#212230,#212231,#212232,#212233,#212234,#212235,#212236),
 .UNSPECIFIED.,.F.,.F.,(4,3,3,3,3,3,3,3,3,3,3,3,3,4),(0.,6.845642507945E-5,
0.00013828840658994,0.000205407478922911,0.000256966021225852,0.000257101146970265,
0.000271589374668169,0.000352213067613375,0.000388398097499794,0.000404123622054886,
0.000459162957997708,0.000486682625969119,0.000500442459954824,0.00051420229394053),
 .UNSPECIFIED.);
#4771=B_SPLINE_CURVE_WITH_KNOTS('',3,(#212240,#212241,#212242,#212243,#212244,
#212245,#212246,#212247,#212248,#212249,#212250,#212251,#212252,#212253,
#212254,#212255,#212256,#212257,#212258,#212259,#212260,#212261,#212262,
#212263,#212264,#212265,#212266,#212267,#212268,#212269,#212270,#212271,
#212272,#212273,#212274,#212275,#212276,#212277,#212278,#212279,#212280,
#212281,#212282),.UNSPECIFIED.,.F.,.F.,(4,3,3,3,3,3,3,3,3,3,3,3,3,3,4),
(0.,1.12890698065816E-5,7.65259667026669E-5,0.000102837507928515,0.000112544869199256,
0.000130746171581896,0.000194450729921135,0.000226303009090754,0.000242229148675564,
0.000258155288260373,0.000258291104876517,0.000327654633613867,0.000399363990833934,
0.0004697092851882,0.000516310576520747),.UNSPECIFIED.);
#4772=B_SPLINE_CURVE_WITH_KNOTS('',3,(#212290,#212291,#212292,#212293,#212294,
#212295,#212296,#212297,#212298,#212299,#212300,#212301,#212302,#212303,
#212304,#212305,#212306,#212307,#212308,#212309,#212310,#212311,#212312,
#212313,#212314,#212315,#212316,#212317,#212318,#212319,#212320,#212321,
#212322,#212323,#212324,#212325,#212326,#212327,#212328,#212329),
 .UNSPECIFIED.,.F.,.F.,(4,3,3,3,3,3,3,3,3,3,3,3,3,4),(0.,6.84564250866856E-5,
0.000138288406604513,0.000205407478944171,0.00025696602122585,0.00025710114697026,
0.000271589374668166,0.000352213067614554,0.00038839809749983,0.000404123622054916,
0.000459162957997718,0.000486682625969119,0.00050044245995482,0.00051420229394052),
 .UNSPECIFIED.);
#4773=B_SPLINE_CURVE_WITH_KNOTS('',3,(#212333,#212334,#212335,#212336,#212337,
#212338,#212339,#212340,#212341,#212342,#212343,#212344,#212345,#212346,
#212347,#212348,#212349,#212350,#212351,#212352,#212353,#212354,#212355,
#212356,#212357,#212358,#212359,#212360,#212361,#212362,#212363,#212364,
#212365,#212366,#212367,#212368,#212369,#212370,#212371,#212372,#212373,
#212374,#212375),.UNSPECIFIED.,.F.,.F.,(4,3,3,3,3,3,3,3,3,3,3,3,3,3,4),
(0.,1.12890698065806E-5,7.65259667141636E-5,0.000102837507928481,0.000112544869199224,
0.000130746171581867,0.000194450729921119,0.000226303009090746,0.000242229148675559,
0.000258155288260372,0.000258291104876518,0.000327654633616041,0.000399363990838671,
0.000469709285194909,0.000516310576520743),.UNSPECIFIED.);
#4774=B_SPLINE_CURVE_WITH_KNOTS('',3,(#212383,#212384,#212385,#212386,#212387,
#212388,#212389,#212390,#212391,#212392,#212393,#212394,#212395,#212396,
#212397,#212398,#212399,#212400,#212401,#212402,#212403,#212404,#212405,
#212406,#212407,#212408,#212409,#212410,#212411,#212412,#212413,#212414,
#212415,#212416,#212417,#212418,#212419,#212420,#212421,#212422),
 .UNSPECIFIED.,.F.,.F.,(4,3,3,3,3,3,3,3,3,3,3,3,3,4),(0.,6.84564250774396E-5,
0.000138288406586533,0.000205407478919854,0.000256966021225855,0.00025710114697026,
0.000271589374668168,0.000352213067602211,0.000388398097499803,0.000404123622054893,
0.000459162957997706,0.000486682625969113,0.000500442459954816,0.000514202293940519),
 .UNSPECIFIED.);
#4775=B_SPLINE_CURVE_WITH_KNOTS('',3,(#212426,#212427,#212428,#212429,#212430,
#212431,#212432,#212433,#212434,#212435,#212436,#212437,#212438,#212439,
#212440,#212441,#212442,#212443,#212444,#212445,#212446,#212447,#212448,
#212449,#212450,#212451,#212452,#212453,#212454,#212455,#212456,#212457,
#212458,#212459,#212460,#212461,#212462,#212463,#212464,#212465,#212466,
#212467,#212468),.UNSPECIFIED.,.F.,.F.,(4,3,3,3,3,3,3,3,3,3,3,3,3,3,4),
(0.,1.12890698065791E-5,7.65259667026007E-5,0.000102837507928491,0.000112544869199234,
0.000130746171581876,0.000194450729921125,0.00022630300909075,0.000242229148675562,
0.000258155288260374,0.000258291104876513,0.000327654633618617,0.000399363990843893,
0.000469709285202695,0.000516310576520748),.UNSPECIFIED.);
#4776=B_SPLINE_CURVE_WITH_KNOTS('',3,(#212476,#212477,#212478,#212479,#212480,
#212481,#212482,#212483,#212484,#212485,#212486,#212487,#212488,#212489,
#212490,#212491,#212492,#212493,#212494,#212495,#212496,#212497,#212498,
#212499,#212500,#212501,#212502,#212503,#212504,#212505,#212506,#212507,
#212508,#212509,#212510,#212511,#212512,#212513,#212514,#212515),
 .UNSPECIFIED.,.F.,.F.,(4,3,3,3,3,3,3,3,3,3,3,3,3,4),(0.,6.84564250846693E-5,
0.000138288406600395,0.000205407478938273,0.000256966021225847,0.000257101146970259,
0.000271589374668162,0.000352213067606228,0.000388398097499803,0.000404123622054892,
0.000459162957997705,0.000486682625969112,0.000500442459954815,0.000514202293940518),
 .UNSPECIFIED.);
#4777=B_SPLINE_CURVE_WITH_KNOTS('',3,(#212519,#212520,#212521,#212522,#212523,
#212524,#212525,#212526,#212527,#212528,#212529,#212530,#212531,#212532,
#212533,#212534,#212535,#212536,#212537,#212538,#212539,#212540,#212541,
#212542,#212543,#212544,#212545,#212546,#212547,#212548,#212549,#212550,
#212551,#212552,#212553,#212554,#212555,#212556,#212557,#212558,#212559,
#212560,#212561),.UNSPECIFIED.,.F.,.F.,(4,3,3,3,3,3,3,3,3,3,3,3,3,3,4),
(0.,1.12890698065812E-5,7.65259667018894E-5,0.000102837507928503,0.000112544869199245,
0.000130746171581885,0.000194450729921128,0.000226303009090749,0.00024222914867556,
0.00025815528826037,0.000258291104876506,0.000327654633607904,0.000399363990821826,
0.000469709285170662,0.000516310576520741),.UNSPECIFIED.);
#4778=B_SPLINE_CURVE_WITH_KNOTS('',3,(#212569,#212570,#212571,#212572,#212573,
#212574,#212575,#212576,#212577,#212578,#212579,#212580,#212581,#212582,
#212583,#212584,#212585,#212586,#212587,#212588,#212589,#212590,#212591,
#212592,#212593,#212594,#212595,#212596,#212597,#212598,#212599,#212600,
#212601,#212602,#212603,#212604,#212605,#212606,#212607,#212608),
 .UNSPECIFIED.,.F.,.F.,(4,3,3,3,3,3,3,3,3,3,3,3,3,4),(1.30104260698261E-18,
6.84564250830632E-5,0.000138288406597626,0.000205407478935301,0.000256966021225847,
0.000257101146970268,0.000271589374668169,0.00035221306760621,0.00038839809749974,
0.000404123622054839,0.000459162957997687,0.000486682625969111,0.000500442459954823,
0.000514202293940535),.UNSPECIFIED.);
#4779=B_SPLINE_CURVE_WITH_KNOTS('',3,(#212612,#212613,#212614,#212615,#212616,
#212617,#212618,#212619,#212620,#212621,#212622,#212623,#212624,#212625,
#212626,#212627,#212628,#212629,#212630,#212631,#212632,#212633,#212634,
#212635,#212636,#212637,#212638,#212639,#212640,#212641,#212642,#212643,
#212644,#212645,#212646,#212647,#212648,#212649,#212650,#212651,#212652,
#212653,#212654),.UNSPECIFIED.,.F.,.F.,(4,3,3,3,3,3,3,3,3,3,3,3,3,3,4),
(0.,1.12890698065819E-5,7.65259666993655E-5,0.000102837507928517,0.000112544869199258,
0.000130746171581898,0.000194450729921138,0.000226303009090758,0.000242229148675569,
0.000258155288260379,0.000258291104876534,0.000327654633615767,0.000399363990838623,
0.00046970928519652,0.000516310576520757),.UNSPECIFIED.);
#4780=B_SPLINE_CURVE_WITH_KNOTS('',3,(#212662,#212663,#212664,#212665,#212666,
#212667,#212668,#212669,#212670,#212671,#212672,#212673,#212674,#212675,
#212676,#212677,#212678,#212679,#212680,#212681,#212682,#212683,#212684,
#212685,#212686,#212687,#212688,#212689,#212690,#212691,#212692,#212693,
#212694,#212695,#212696,#212697,#212698,#212699,#212700,#212701),
 .UNSPECIFIED.,.F.,.F.,(4,3,3,3,3,3,3,3,3,3,3,3,3,4),(1.73472347597681E-18,
6.84564250816081E-5,0.000138288406594168,0.000205407478929045,0.000256966021225858,
0.000257101146970264,0.000271589374668166,0.000352213067603754,0.000388398097499799,
0.000404123622054889,0.000459162957997708,0.000486682625969117,0.000500442459954821,
0.000514202293940526),.UNSPECIFIED.);
#4781=B_SPLINE_CURVE_WITH_KNOTS('',3,(#212705,#212706,#212707,#212708,#212709,
#212710,#212711,#212712,#212713,#212714,#212715,#212716,#212717,#212718,
#212719,#212720,#212721,#212722,#212723,#212724,#212725,#212726,#212727,
#212728,#212729,#212730,#212731,#212732,#212733,#212734,#212735,#212736,
#212737,#212738,#212739,#212740,#212741,#212742,#212743,#212744,#212745,
#212746,#212747),.UNSPECIFIED.,.F.,.F.,(4,3,3,3,3,3,3,3,3,3,3,3,3,3,4),
(0.,1.12890698065796E-5,7.65259667013587E-5,0.000102837507928479,0.000112544869199222,
0.000130746171581866,0.00019445072992112,0.000226303009090747,0.00024222914867556,
0.000258155288260373,0.000258291104876525,0.000327654633618632,0.000399363990844032,
0.000469709285203426,0.000516310576520747),.UNSPECIFIED.);
#4782=B_SPLINE_CURVE_WITH_KNOTS('',3,(#212755,#212756,#212757,#212758,#212759,
#212760,#212761,#212762,#212763,#212764,#212765,#212766,#212767,#212768,
#212769,#212770,#212771,#212772,#212773,#212774,#212775,#212776,#212777,
#212778,#212779,#212780,#212781,#212782,#212783,#212784,#212785,#212786,
#212787,#212788,#212789,#212790,#212791,#212792,#212793,#212794),
 .UNSPECIFIED.,.F.,.F.,(4,3,3,3,3,3,3,3,3,3,3,3,3,4),(3.03576608295941E-18,
6.84564250824445E-5,0.000138288406596601,0.000205407478934739,0.000256966021225856,
0.000257101146970265,0.000271589374668165,0.000352213067598913,0.000388398097499742,
0.00040412362205484,0.000459162957997684,0.000486682625969106,0.000500442459954816,
0.000514202293940527),.UNSPECIFIED.);
#4783=B_SPLINE_CURVE_WITH_KNOTS('',3,(#212798,#212799,#212800,#212801,#212802,
#212803,#212804,#212805,#212806,#212807,#212808,#212809,#212810,#212811,
#212812,#212813,#212814,#212815,#212816,#212817,#212818,#212819,#212820,
#212821,#212822,#212823,#212824,#212825,#212826,#212827,#212828,#212829,
#212830,#212831,#212832,#212833,#212834,#212835,#212836,#212837,#212838,
#212839,#212840),.UNSPECIFIED.,.F.,.F.,(4,3,3,3,3,3,3,3,3,3,3,3,3,3,4),
(0.,1.12890698065835E-5,7.65259667091678E-5,0.000102837507928531,0.000112544869199271,
0.000130746171581909,0.000194450729921141,0.000226303009090757,0.000242229148675566,
0.000258155288260374,0.000258291104876515,0.000327654633617367,0.000399363990841117,
0.000469709285198328,0.000516310576520747),.UNSPECIFIED.);
#4784=B_SPLINE_CURVE_WITH_KNOTS('',3,(#212848,#212849,#212850,#212851,#212852,
#212853,#212854,#212855,#212856,#212857,#212858,#212859,#212860,#212861,
#212862,#212863,#212864,#212865,#212866,#212867,#212868,#212869,#212870,
#212871,#212872,#212873,#212874,#212875,#212876,#212877,#212878,#212879,
#212880,#212881,#212882,#212883,#212884,#212885,#212886,#212887),
 .UNSPECIFIED.,.F.,.F.,(4,3,3,3,3,3,3,3,3,3,3,3,3,4),(0.,6.84564250852912E-5,
0.000138288406602005,0.000205407478941458,0.000256966021225849,0.000257101146970268,
0.000271589374668176,0.000352213067603525,0.000388398097499865,0.000404123622054949,
0.000459162957997742,0.000486682625969139,0.000500442459954838,0.000514202293940536),
 .UNSPECIFIED.);
#4785=B_SPLINE_CURVE_WITH_KNOTS('',3,(#212891,#212892,#212893,#212894,#212895,
#212896,#212897,#212898,#212899,#212900,#212901,#212902,#212903,#212904,
#212905,#212906,#212907,#212908,#212909,#212910,#212911,#212912,#212913,
#212914,#212915,#212916,#212917,#212918,#212919,#212920,#212921,#212922,
#212923,#212924,#212925,#212926,#212927,#212928,#212929,#212930,#212931,
#212932,#212933),.UNSPECIFIED.,.F.,.F.,(4,3,3,3,3,3,3,3,3,3,3,3,3,3,4),
(0.,1.12890698065827E-5,7.65259667068948E-5,0.00010283750792852,0.00011254486919926,
0.000130746171581899,0.000194450729921134,0.000226303009090752,0.000242229148675561,
0.000258155288260369,0.000258291104876524,0.000327654633614918,0.000399363990836254,
0.000469709285191718,0.000516310576520739),.UNSPECIFIED.);
#4786=B_SPLINE_CURVE_WITH_KNOTS('',3,(#212941,#212942,#212943,#212944,#212945,
#212946,#212947,#212948,#212949,#212950,#212951,#212952,#212953,#212954,
#212955,#212956,#212957,#212958,#212959,#212960,#212961,#212962,#212963,
#212964,#212965,#212966,#212967,#212968,#212969,#212970,#212971,#212972,
#212973,#212974,#212975,#212976,#212977,#212978,#212979,#212980),
 .UNSPECIFIED.,.F.,.F.,(4,3,3,3,3,3,3,3,3,3,3,3,3,4),(0.,6.84564250828912E-5,
0.000138288406596643,0.000205407478932016,0.000256966021225854,0.000257101146970266,
0.000271589374668171,0.000352213067611571,0.000388398097499799,0.000404123622054891,
0.000459162957997711,0.000486682625969122,0.000500442459954827,0.000514202293940532),
 .UNSPECIFIED.);
#4787=B_SPLINE_CURVE_WITH_KNOTS('',3,(#212984,#212985,#212986,#212987,#212988,
#212989,#212990,#212991,#212992,#212993,#212994,#212995,#212996,#212997,
#212998,#212999,#213000,#213001,#213002,#213003,#213004,#213005,#213006,
#213007,#213008,#213009,#213010,#213011,#213012,#213013,#213014,#213015,
#213016,#213017,#213018,#213019,#213020,#213021,#213022,#213023,#213024,
#213025,#213026),.UNSPECIFIED.,.F.,.F.,(4,3,3,3,3,3,3,3,3,3,3,3,3,3,4),
(0.,1.12890698065862E-5,7.6525966702336E-5,0.000102837507928534,0.000112544869199274,
0.000130746171581911,0.000194450729921141,0.000226303009090756,0.000242229148675563,
0.00025815528826037,0.000258291104876527,0.000327654633615046,0.000399363990836708,
0.000469709285192809,0.000516310576520741),.UNSPECIFIED.);
#4788=B_SPLINE_CURVE_WITH_KNOTS('',3,(#213034,#213035,#213036,#213037,#213038,
#213039,#213040,#213041,#213042,#213043,#213044,#213045,#213046,#213047,
#213048,#213049,#213050,#213051,#213052,#213053,#213054,#213055,#213056,
#213057,#213058,#213059,#213060,#213061,#213062,#213063,#213064,#213065,
#213066,#213067,#213068,#213069,#213070,#213071,#213072,#213073),
 .UNSPECIFIED.,.F.,.F.,(4,3,3,3,3,3,3,3,3,3,3,3,3,4),(0.,6.84564250856532E-5,
0.000138288406601763,0.000205407478938914,0.000256966021225856,0.000257101146970268,
0.000271589374668171,0.00035221306760409,0.000388398097499817,0.000404123622054907,
0.000459162957997721,0.000486682625969128,0.000500442459954832,0.000514202293940535),
 .UNSPECIFIED.);
#4789=B_SPLINE_CURVE_WITH_KNOTS('',3,(#213077,#213078,#213079,#213080,#213081,
#213082,#213083,#213084,#213085,#213086,#213087,#213088,#213089,#213090,
#213091,#213092,#213093,#213094,#213095,#213096,#213097,#213098,#213099,
#213100,#213101,#213102,#213103,#213104,#213105,#213106,#213107,#213108,
#213109,#213110,#213111,#213112,#213113,#213114,#213115,#213116,#213117,
#213118,#213119),.UNSPECIFIED.,.F.,.F.,(4,3,3,3,3,3,3,3,3,3,3,3,3,3,4),
(0.,1.12890698065867E-5,7.65259667130106E-5,0.000102837507928551,0.00011254486919929,
0.000130746171581926,0.000194450729921151,0.000226303009090763,0.00024222914867557,
0.000258155288260376,0.000258291104876518,0.000327654633617211,0.000399363990841065,
0.000469709285198404,0.000516310576520752),.UNSPECIFIED.);
#4790=B_SPLINE_CURVE_WITH_KNOTS('',3,(#213127,#213128,#213129,#213130,#213131,
#213132,#213133,#213134,#213135,#213136,#213137,#213138,#213139,#213140,
#213141,#213142,#213143,#213144,#213145,#213146,#213147,#213148,#213149,
#213150,#213151,#213152,#213153,#213154,#213155,#213156,#213157,#213158,
#213159,#213160,#213161,#213162,#213163,#213164,#213165,#213166),
 .UNSPECIFIED.,.F.,.F.,(4,3,3,3,3,3,3,3,3,3,3,3,3,4),(0.,6.84564250819788E-5,
0.000138288406594927,0.000205407478930393,0.000256966021225853,0.000257101146970261,
0.000271589374668166,0.000352213067606589,0.000388398097499793,0.000404123622054884,
0.000459162957997703,0.000486682625969113,0.000500442459954818,0.000514202293940523),
 .UNSPECIFIED.);
#4791=B_SPLINE_CURVE_WITH_KNOTS('',3,(#213170,#213171,#213172,#213173,#213174,
#213175,#213176,#213177,#213178,#213179,#213180,#213181,#213182,#213183,
#213184,#213185,#213186,#213187,#213188,#213189,#213190,#213191,#213192,
#213193,#213194,#213195,#213196,#213197,#213198,#213199,#213200,#213201,
#213202,#213203,#213204,#213205,#213206,#213207,#213208,#213209,#213210,
#213211,#213212),.UNSPECIFIED.,.F.,.F.,(4,3,3,3,3,3,3,3,3,3,3,3,3,3,4),
(0.,1.12890698065856E-5,7.65259667056268E-5,0.000102837507928536,0.000112544869199275,
0.000130746171581911,0.000194450729921138,0.000226303009090751,0.000242229148675558,
0.000258155288260364,0.000258291104876502,0.000327654633618074,0.000399363990842774,
0.00046970928520123,0.000516310576520728),.UNSPECIFIED.);
#4792=B_SPLINE_CURVE_WITH_KNOTS('',3,(#213220,#213221,#213222,#213223,#213224,
#213225,#213226,#213227,#213228,#213229,#213230,#213231,#213232,#213233,
#213234,#213235,#213236,#213237,#213238,#213239,#213240,#213241,#213242,
#213243,#213244,#213245,#213246,#213247,#213248,#213249,#213250,#213251,
#213252,#213253,#213254,#213255,#213256,#213257,#213258,#213259),
 .UNSPECIFIED.,.F.,.F.,(4,3,3,3,3,3,3,3,3,3,3,3,3,4),(0.,6.84564250843941E-5,
0.000138288406600047,0.000205407478938544,0.000256966021225849,0.000257101146970261,
0.000271589374668161,0.000352213067598837,0.000388398097499768,0.000404123622054862,
0.000459162957997692,0.000486682625969107,0.000500442459954815,0.000514202293940522),
 .UNSPECIFIED.);
#4793=B_SPLINE_CURVE_WITH_KNOTS('',3,(#213263,#213264,#213265,#213266,#213267,
#213268,#213269,#213270,#213271,#213272,#213273,#213274,#213275,#213276,
#213277,#213278,#213279,#213280,#213281,#213282,#213283,#213284,#213285,
#213286,#213287,#213288,#213289,#213290,#213291,#213292,#213293,#213294,
#213295,#213296,#213297,#213298,#213299,#213300,#213301,#213302,#213303,
#213304,#213305),.UNSPECIFIED.,.F.,.F.,(4,3,3,3,3,3,3,3,3,3,3,3,3,3,4),
(0.,1.12890698065839E-5,7.65259667039472E-5,0.000102837507928521,0.000112544869199262,
0.000130746171581902,0.00019445072992114,0.000226303009090759,0.000242229148675569,
0.000258155288260379,0.000258291104876519,0.00032765463361463,0.000399363990835635,
0.000469709285190714,0.000516310576520757),.UNSPECIFIED.);
#4794=B_SPLINE_CURVE_WITH_KNOTS('',3,(#213312,#213313,#213314,#213315,#213316,
#213317,#213318,#213319,#213320,#213321,#213322,#213323,#213324,#213325,
#213326,#213327,#213328,#213329,#213330,#213331,#213332,#213333,#213334,
#213335,#213336,#213337,#213338,#213339,#213340,#213341,#213342,#213343,
#213344,#213345,#213346,#213347,#213348,#213349,#213350,#213351),
 .UNSPECIFIED.,.F.,.F.,(4,3,3,3,3,3,3,3,3,3,3,3,3,4),(0.,6.84564250787631E-5,
0.000138288406588445,0.000205407478920956,0.000256966021225842,0.000257101146970262,
0.000271589374668168,0.00035221306760281,0.000388398097499837,0.000404123622054923,
0.000459162957997723,0.000486682625969124,0.000500442459954824,0.000514202293940524),
 .UNSPECIFIED.);
#4795=B_SPLINE_CURVE_WITH_KNOTS('',3,(#213354,#213355,#213356,#213357,#213358,
#213359,#213360,#213361,#213362,#213363,#213364,#213365,#213366,#213367,
#213368,#213369,#213370,#213371,#213372,#213373,#213374,#213375,#213376,
#213377,#213378,#213379,#213380,#213381,#213382,#213383,#213384,#213385,
#213386,#213387,#213388,#213389,#213390,#213391,#213392,#213393,#213394,
#213395,#213396),.UNSPECIFIED.,.F.,.F.,(4,3,3,3,3,3,3,3,3,3,3,3,3,3,4),
(0.,1.1289069806579E-5,7.65259666957119E-5,0.000102837507928486,0.000112544869199229,
0.000130746171581871,0.00019445072992112,0.000226303009090744,0.000242229148675556,
0.000258155288260368,0.000258291104876506,0.000327654633618157,0.000399363990842572,
0.000469709285200546,0.000516310576520737),.UNSPECIFIED.);
#4796=B_SPLINE_CURVE_WITH_KNOTS('',3,(#213404,#213405,#213406,#213407,#213408,
#213409,#213410,#213411,#213412,#213413,#213414,#213415,#213416,#213417,
#213418,#213419,#213420,#213421,#213422,#213423,#213424,#213425,#213426,
#213427,#213428,#213429,#213430,#213431,#213432,#213433,#213434,#213435,
#213436,#213437,#213438,#213439,#213440,#213441,#213442,#213443),
 .UNSPECIFIED.,.F.,.F.,(4,3,3,3,3,3,3,3,3,3,3,3,3,4),(4.33680868994202E-19,
6.8456425087802E-5,0.000138288406606736,0.000205407478947457,0.00025696602122585,
0.00025710114697026,0.000271589374668168,0.000352213067608876,0.000388398097499855,
0.000404123622054938,0.000459162957997729,0.000486682625969124,0.000500442459954822,
0.00051420229394052),.UNSPECIFIED.);
#4797=B_SPLINE_CURVE_WITH_KNOTS('',3,(#213447,#213448,#213449,#213450,#213451,
#213452,#213453,#213454,#213455,#213456,#213457,#213458,#213459,#213460,
#213461,#213462,#213463,#213464,#213465,#213466,#213467,#213468,#213469,
#213470,#213471,#213472,#213473,#213474,#213475,#213476,#213477,#213478,
#213479,#213480,#213481,#213482,#213483,#213484,#213485,#213486,#213487,
#213488,#213489),.UNSPECIFIED.,.F.,.F.,(4,3,3,3,3,3,3,3,3,3,3,3,3,3,4),
(0.,1.12890698065821E-5,7.65259666989574E-5,0.000102837507928512,0.000112544869199253,
0.000130746171581893,0.000194450729921131,0.00022630300909075,0.000242229148675559,
0.000258155288260368,0.000258291104876505,0.000327654633622185,0.000399363990850742,
0.000469709285212212,0.000516310576520737),.UNSPECIFIED.);
#4798=B_SPLINE_CURVE_WITH_KNOTS('',3,(#213497,#213498,#213499,#213500,#213501,
#213502,#213503,#213504,#213505,#213506,#213507,#213508,#213509,#213510,
#213511,#213512,#213513,#213514,#213515,#213516,#213517,#213518,#213519,
#213520,#213521,#213522,#213523,#213524,#213525,#213526,#213527,#213528,
#213529,#213530,#213531,#213532,#213533,#213534,#213535,#213536),
 .UNSPECIFIED.,.F.,.F.,(4,3,3,3,3,3,3,3,3,3,3,3,3,4),(0.,6.84564250781753E-5,
0.000138288406587289,0.000205407478919208,0.00025696602122585,0.000257101146970262,
0.000271589374668164,0.000352213067607333,0.00038839809749979,0.000404123622054882,
0.000459162957997703,0.000486682625969114,0.000500442459954819,0.000514202293940525),
 .UNSPECIFIED.);
#4799=B_SPLINE_CURVE_WITH_KNOTS('',3,(#213540,#213541,#213542,#213543,#213544,
#213545,#213546,#213547,#213548,#213549,#213550,#213551,#213552,#213553,
#213554,#213555,#213556,#213557,#213558,#213559,#213560,#213561,#213562,
#213563,#213564,#213565,#213566,#213567,#213568,#213569,#213570,#213571,
#213572,#213573,#213574,#213575,#213576,#213577,#213578,#213579,#213580,
#213581,#213582),.UNSPECIFIED.,.F.,.F.,(4,3,3,3,3,3,3,3,3,3,3,3,3,3,4),
(0.,1.12890698065806E-5,7.65259667054612E-5,0.000102837507928489,0.000112544869199231,
0.000130746171581873,0.000194450729921119,0.000226303009090741,0.000242229148675553,
0.000258155288260364,0.000258291104876508,0.000327654633618402,0.000399363990843321,
0.000469709285201685,0.000516310576520728),.UNSPECIFIED.);
#4800=B_SPLINE_CURVE_WITH_KNOTS('',3,(#213590,#213591,#213592,#213593,#213594,
#213595,#213596,#213597,#213598,#213599,#213600,#213601,#213602,#213603,
#213604,#213605,#213606,#213607,#213608,#213609,#213610,#213611,#213612,
#213613,#213614,#213615,#213616,#213617,#213618,#213619,#213620,#213621,
#213622,#213623,#213624,#213625,#213626,#213627,#213628,#213629),
 .UNSPECIFIED.,.F.,.F.,(4,3,3,3,3,3,3,3,3,3,3,3,3,4),(4.33680868994202E-19,
6.84564250831933E-5,0.000138288406597582,0.000205407478934626,0.000256966021225843,
0.000257101146970263,0.000271589374668168,0.000352213067601041,0.00038839809749985,
0.000404123622054935,0.00045916295799773,0.000486682625969128,0.000500442459954826,
0.000514202293940525),.UNSPECIFIED.);
#4801=B_SPLINE_CURVE_WITH_KNOTS('',3,(#213633,#213634,#213635,#213636,#213637,
#213638,#213639,#213640,#213641,#213642,#213643,#213644,#213645,#213646,
#213647,#213648,#213649,#213650,#213651,#213652,#213653,#213654,#213655,
#213656,#213657,#213658,#213659,#213660,#213661,#213662,#213663,#213664,
#213665,#213666,#213667,#213668,#213669,#213670,#213671,#213672,#213673,
#213674,#213675),.UNSPECIFIED.,.F.,.F.,(4,3,3,3,3,3,3,3,3,3,3,3,3,3,4),
(0.,1.12890698065816E-5,7.6525966705804E-5,0.000102837507928503,0.000112544869199245,
0.000130746171581886,0.000194450729921129,0.000226303009090751,0.000242229148675562,
0.000258155288260373,0.000258291104876505,0.000327654633620337,0.000399363990847408,
0.000469709285207948,0.000516310576520746),.UNSPECIFIED.);
#4802=B_SPLINE_CURVE_WITH_KNOTS('',3,(#213683,#213684,#213685,#213686,#213687,
#213688,#213689,#213690,#213691,#213692,#213693,#213694,#213695,#213696,
#213697,#213698,#213699,#213700,#213701,#213702,#213703,#213704,#213705,
#213706,#213707,#213708,#213709,#213710,#213711,#213712,#213713,#213714,
#213715,#213716,#213717,#213718,#213719,#213720,#213721,#213722),
 .UNSPECIFIED.,.F.,.F.,(4,3,3,3,3,3,3,3,3,3,3,3,3,4),(1.30104260698261E-18,
6.8456425086901E-5,0.000138288406605303,0.000205407478945984,0.00025696602122585,
0.000257101146970262,0.000271589374668163,0.000352213067612747,0.000388398097499783,
0.000404123622054875,0.000459162957997699,0.000486682625969111,0.000500442459954817,
0.000514202293940523),.UNSPECIFIED.);
#4803=B_SPLINE_CURVE_WITH_KNOTS('',3,(#213726,#213727,#213728,#213729,#213730,
#213731,#213732,#213733,#213734,#213735,#213736,#213737,#213738,#213739,
#213740,#213741,#213742,#213743,#213744,#213745,#213746,#213747,#213748,
#213749,#213750,#213751,#213752,#213753,#213754,#213755,#213756,#213757,
#213758,#213759,#213760,#213761,#213762,#213763,#213764,#213765,#213766,
#213767,#213768),.UNSPECIFIED.,.F.,.F.,(4,3,3,3,3,3,3,3,3,3,3,3,3,3,4),
(0.,1.12890698065817E-5,7.65259667124228E-5,0.000102837507928514,0.000112544869199255,
0.000130746171581895,0.000194450729921135,0.000226303009090755,0.000242229148675565,
0.000258155288260375,0.000258291104876506,0.000327654633614057,0.000399363990834877,
0.00046970928519008,0.000516310576520749),.UNSPECIFIED.);
#4804=B_SPLINE_CURVE_WITH_KNOTS('',3,(#213776,#213777,#213778,#213779,#213780,
#213781,#213782,#213783,#213784,#213785,#213786,#213787,#213788,#213789,
#213790,#213791,#213792,#213793,#213794,#213795,#213796,#213797,#213798,
#213799,#213800,#213801,#213802,#213803,#213804,#213805,#213806,#213807,
#213808,#213809,#213810,#213811,#213812,#213813,#213814,#213815),
 .UNSPECIFIED.,.F.,.F.,(4,3,3,3,3,3,3,3,3,3,3,3,3,4),(0.,6.8456425084337E-5,
0.000138288406599689,0.000205407478937187,0.000256966021225854,0.000257101146970268,
0.00027158937466817,0.000352213067599072,0.000388398097499823,0.000404123622054912,
0.000459162957997724,0.00048668262596913,0.000500442459954833,0.000514202293940536),
 .UNSPECIFIED.);
#4805=B_SPLINE_CURVE_WITH_KNOTS('',3,(#213819,#213820,#213821,#213822,#213823,
#213824,#213825,#213826,#213827,#213828,#213829,#213830,#213831,#213832,
#213833,#213834,#213835,#213836,#213837,#213838,#213839,#213840,#213841,
#213842,#213843,#213844,#213845,#213846,#213847,#213848,#213849,#213850,
#213851,#213852,#213853,#213854,#213855,#213856,#213857,#213858,#213859,
#213860,#213861),.UNSPECIFIED.,.F.,.F.,(4,3,3,3,3,3,3,3,3,3,3,3,3,3,4),
(0.,1.12890698065782E-5,7.65259667090296E-5,0.0001028375079285,0.000112544869199242,
0.000130746171581883,0.000194450729921127,0.00022630300909075,0.000242229148675561,
0.000258155288260372,0.000258291104876505,0.000327654633625998,0.00039936399085858,
0.000469709285223216,0.000516310576520744),.UNSPECIFIED.);
#4806=B_SPLINE_CURVE_WITH_KNOTS('',3,(#213869,#213870,#213871,#213872,#213873,
#213874,#213875,#213876,#213877,#213878,#213879,#213880,#213881,#213882,
#213883,#213884,#213885,#213886,#213887,#213888,#213889,#213890,#213891,
#213892,#213893,#213894,#213895,#213896,#213897,#213898,#213899,#213900,
#213901,#213902,#213903,#213904,#213905,#213906,#213907,#213908),
 .UNSPECIFIED.,.F.,.F.,(4,3,3,3,3,3,3,3,3,3,3,3,3,4),(8.67361737988404E-19,
6.84564250816429E-5,0.000138288406594391,0.000205407478929637,0.000256966021225841,
0.000257101146970264,0.000271589374668172,0.000352213067612495,0.000388398097499806,
0.000404123622054896,0.000459162957997711,0.000486682625969119,0.000500442459954823,
0.000514202293940526),.UNSPECIFIED.);
#4807=B_SPLINE_CURVE_WITH_KNOTS('',3,(#213912,#213913,#213914,#213915,#213916,
#213917,#213918,#213919,#213920,#213921,#213922,#213923,#213924,#213925,
#213926,#213927,#213928,#213929,#213930,#213931,#213932,#213933,#213934,
#213935,#213936,#213937,#213938,#213939,#213940,#213941,#213942,#213943,
#213944,#213945,#213946,#213947,#213948,#213949,#213950,#213951,#213952,
#213953,#213954),.UNSPECIFIED.,.F.,.F.,(4,3,3,3,3,3,3,3,3,3,3,3,3,3,4),
(0.,1.12890698065835E-5,7.6525966723323E-5,0.000102837507928538,0.000112544869199278,
0.000130746171581915,0.000194450729921145,0.00022630300909076,0.000242229148675568,
0.000258155288260375,0.000258291104876509,0.000327654633610471,0.000399363990827954,
0.000469709285180224,0.000516310576520751),.UNSPECIFIED.);
#4808=B_SPLINE_CURVE_WITH_KNOTS('',3,(#213962,#213963,#213964,#213965,#213966,
#213967,#213968,#213969,#213970,#213971,#213972,#213973,#213974,#213975,
#213976,#213977,#213978,#213979,#213980,#213981,#213982,#213983,#213984,
#213985,#213986,#213987,#213988,#213989,#213990,#213991,#213992,#213993,
#213994,#213995,#213996,#213997,#213998,#213999,#214000,#214001),
 .UNSPECIFIED.,.F.,.F.,(4,3,3,3,3,3,3,3,3,3,3,3,3,4),(0.,6.8456425088049E-5,
0.00013828840660642,0.000205407478945175,0.00025696602122584,0.000257101146970266,
0.000271589374668167,0.000352213067609995,0.000388398097499859,0.000404123622054943,
0.000459162957997738,0.000486682625969135,0.000500442459954834,0.000514202293940532),
 .UNSPECIFIED.);
#4809=B_SPLINE_CURVE_WITH_KNOTS('',3,(#214005,#214006,#214007,#214008,#214009,
#214010,#214011,#214012,#214013,#214014,#214015,#214016,#214017,#214018,
#214019,#214020,#214021,#214022,#214023,#214024,#214025,#214026,#214027,
#214028,#214029,#214030,#214031,#214032,#214033,#214034,#214035,#214036,
#214037,#214038,#214039,#214040,#214041,#214042,#214043,#214044,#214045,
#214046,#214047),.UNSPECIFIED.,.F.,.F.,(4,3,3,3,3,3,3,3,3,3,3,3,3,3,4),
(0.,1.12890698065781E-5,7.65259667000974E-5,0.000102837507928479,0.000112544869199222,
0.000130746171581865,0.000194450729921117,0.000226303009090743,0.000242229148675556,
0.000258155288260369,0.000258291104876513,0.000327654633621327,0.000399363990848474,
0.000469709285207863,0.000516310576520738),.UNSPECIFIED.);
#4810=B_SPLINE_CURVE_WITH_KNOTS('',3,(#214055,#214056,#214057,#214058,#214059,
#214060,#214061,#214062,#214063,#214064,#214065,#214066,#214067,#214068,
#214069,#214070,#214071,#214072,#214073,#214074,#214075,#214076,#214077,
#214078,#214079,#214080,#214081,#214082,#214083,#214084,#214085,#214086,
#214087,#214088,#214089,#214090,#214091,#214092,#214093,#214094),
 .UNSPECIFIED.,.F.,.F.,(4,3,3,3,3,3,3,3,3,3,3,3,3,4),(0.,6.84564250764968E-5,
0.000138288406584722,0.000205407478917204,0.000256966021225873,0.000257101146970265,
0.000271589374668165,0.000352213067601251,0.000388398097499829,0.000404123622054916,
0.000459162957997723,0.000486682625969127,0.000500442459954828,0.00051420229394053),
 .UNSPECIFIED.);
#4811=B_SPLINE_CURVE_WITH_KNOTS('',3,(#214098,#214099,#214100,#214101,#214102,
#214103,#214104,#214105,#214106,#214107,#214108,#214109,#214110,#214111,
#214112,#214113,#214114,#214115,#214116,#214117,#214118,#214119,#214120,
#214121,#214122,#214123,#214124,#214125,#214126,#214127,#214128,#214129,
#214130,#214131,#214132,#214133,#214134,#214135,#214136,#214137,#214138,
#214139,#214140),.UNSPECIFIED.,.F.,.F.,(4,3,3,3,3,3,3,3,3,3,3,3,3,3,4),
(0.,1.12890698065823E-5,7.6525966699459E-5,0.000102837507928546,0.000112544869199285,
0.000130746171581921,0.000194450729921148,0.000226303009090761,0.000242229148675567,
0.000258155288260374,0.000258291104876522,0.000327654633612774,0.000399363990831956,
0.000469709285185906,0.000516310576520748),.UNSPECIFIED.);
#4812=B_SPLINE_CURVE_WITH_KNOTS('',3,(#214148,#214149,#214150,#214151,#214152,
#214153,#214154,#214155,#214156,#214157,#214158,#214159,#214160,#214161,
#214162,#214163,#214164,#214165,#214166,#214167,#214168,#214169,#214170,
#214171,#214172,#214173,#214174,#214175,#214176,#214177,#214178,#214179,
#214180,#214181,#214182,#214183,#214184,#214185,#214186,#214187),
 .UNSPECIFIED.,.F.,.F.,(4,3,3,3,3,3,3,3,3,3,3,3,3,4),(2.16840434497101E-18,
6.84564250792317E-5,0.000138288406589936,0.000205407478924871,0.000256966021225843,
0.000257101146970267,0.000271589374668169,0.000352213067585113,0.00038839809749978,
0.000404123622054874,0.000459162957997703,0.000486682625969117,0.000500442459954824,
0.000514202293940531),.UNSPECIFIED.);
#4813=B_SPLINE_CURVE_WITH_KNOTS('',3,(#214191,#214192,#214193,#214194,#214195,
#214196,#214197,#214198,#214199,#214200,#214201,#214202,#214203,#214204,
#214205,#214206,#214207,#214208,#214209,#214210,#214211,#214212,#214213,
#214214,#214215,#214216,#214217,#214218,#214219,#214220,#214221,#214222,
#214223,#214224,#214225,#214226,#214227,#214228,#214229,#214230,#214231,
#214232,#214233),.UNSPECIFIED.,.F.,.F.,(4,3,3,3,3,3,3,3,3,3,3,3,3,3,4),
(0.,1.12890698065786E-5,7.65259667078253E-5,0.000102837507928478,0.000112544869199221,
0.000130746171581865,0.00019445072992112,0.000226303009090747,0.000242229148675561,
0.000258155288260374,0.000258291104876519,0.000327654633616867,0.000399363990839437,
0.000469709285194635,0.000516310576520749),.UNSPECIFIED.);
#4814=B_SPLINE_CURVE_WITH_KNOTS('',3,(#214241,#214242,#214243,#214244,#214245,
#214246,#214247,#214248,#214249,#214250,#214251,#214252,#214253,#214254,
#214255,#214256,#214257,#214258,#214259,#214260,#214261,#214262,#214263,
#214264,#214265,#214266,#214267,#214268,#214269,#214270,#214271,#214272,
#214273,#214274,#214275,#214276,#214277,#214278,#214279,#214280),
 .UNSPECIFIED.,.F.,.F.,(4,3,3,3,3,3,3,3,3,3,3,3,3,4),(0.,6.84564250887403E-5,
0.000138288406608633,0.000205407478950316,0.000256966021225859,0.000257101146970265,
0.000271589374668167,0.000352213067601687,0.000388398097499787,0.00040412362205488,
0.000459162957997705,0.000486682625969117,0.000500442459954824,0.00051420229394053),
 .UNSPECIFIED.);
#4815=B_SPLINE_CURVE_WITH_KNOTS('',3,(#214284,#214285,#214286,#214287,#214288,
#214289,#214290,#214291,#214292,#214293,#214294,#214295,#214296,#214297,
#214298,#214299,#214300,#214301,#214302,#214303,#214304,#214305,#214306,
#214307,#214308,#214309,#214310,#214311,#214312,#214313,#214314,#214315,
#214316,#214317,#214318,#214319,#214320,#214321,#214322,#214323,#214324,
#214325,#214326),.UNSPECIFIED.,.F.,.F.,(4,3,3,3,3,3,3,3,3,3,3,3,3,3,4),
(0.,1.12890698065784E-5,7.65259667061265E-5,0.000102837507928456,0.000112544869199201,
0.000130746171581848,0.000194450729921111,0.000226303009090743,0.000242229148675559,
0.000258155288260375,0.000258291104876522,0.000327654633623582,0.000399363990853684,
0.00046970928521631,0.00051631057652075),.UNSPECIFIED.);
#4816=B_SPLINE_CURVE_WITH_KNOTS('',3,(#214334,#214335,#214336,#214337,#214338,
#214339,#214340,#214341,#214342,#214343,#214344,#214345,#214346,#214347,
#214348,#214349,#214350,#214351,#214352,#214353,#214354,#214355,#214356,
#214357,#214358,#214359,#214360,#214361,#214362,#214363,#214364,#214365,
#214366,#214367,#214368,#214369,#214370,#214371,#214372,#214373),
 .UNSPECIFIED.,.F.,.F.,(4,3,3,3,3,3,3,3,3,3,3,3,3,4),(0.,6.84564250746384E-5,
0.000138288406580315,0.000205407478909537,0.000256966021225844,0.000257101146970262,
0.000271589374668164,0.000352213067601251,0.000388398097499803,0.000404123622054893,
0.000459162957997708,0.000486682625969115,0.000500442459954819,0.000514202293940523),
 .UNSPECIFIED.);
#4817=B_SPLINE_CURVE_WITH_KNOTS('',3,(#214377,#214378,#214379,#214380,#214381,
#214382,#214383,#214384,#214385,#214386,#214387,#214388,#214389,#214390,
#214391,#214392,#214393,#214394,#214395,#214396,#214397,#214398,#214399,
#214400,#214401,#214402,#214403,#214404,#214405,#214406,#214407,#214408,
#214409,#214410,#214411,#214412,#214413,#214414,#214415,#214416,#214417,
#214418,#214419),.UNSPECIFIED.,.F.,.F.,(4,3,3,3,3,3,3,3,3,3,3,3,3,3,4),
(0.,1.1289069806584E-5,7.65259667114897E-5,0.000102837507928548,0.000112544869199287,
0.000130746171581922,0.000194450729921144,0.000226303009090756,0.000242229148675561,
0.000258155288260367,0.000258291104876515,0.000327654633614386,0.000399363990835393,
0.00046970928519037,0.000516310576520734),.UNSPECIFIED.);
#4818=B_SPLINE_CURVE_WITH_KNOTS('',3,(#214427,#214428,#214429,#214430,#214431,
#214432,#214433,#214434,#214435,#214436,#214437,#214438,#214439,#214440,
#214441,#214442,#214443,#214444,#214445,#214446,#214447,#214448,#214449,
#214450,#214451,#214452,#214453,#214454,#214455,#214456,#214457,#214458,
#214459,#214460,#214461,#214462,#214463,#214464,#214465,#214466),
 .UNSPECIFIED.,.F.,.F.,(4,3,3,3,3,3,3,3,3,3,3,3,3,4),(0.,6.84564250820019E-5,
0.000138288406594776,0.000205407478930105,0.000256966021225842,0.000257101146970264,
0.000271589374668166,0.000352213067593631,0.000388398097499784,0.000404123622054877,
0.000459162957997702,0.000486682625969115,0.000500442459954821,0.000514202293940528),
 .UNSPECIFIED.);
#4819=B_SPLINE_CURVE_WITH_KNOTS('',3,(#214470,#214471,#214472,#214473,#214474,
#214475,#214476,#214477,#214478,#214479,#214480,#214481,#214482,#214483,
#214484,#214485,#214486,#214487,#214488,#214489,#214490,#214491,#214492,
#214493,#214494,#214495,#214496,#214497,#214498,#214499,#214500,#214501,
#214502,#214503,#214504,#214505,#214506,#214507,#214508,#214509,#214510,
#214511,#214512),.UNSPECIFIED.,.F.,.F.,(4,3,3,3,3,3,3,3,3,3,3,3,3,3,4),
(0.,1.12890698065801E-5,7.65259667059785E-5,0.000102837507928484,0.000112544869199227,
0.000130746171581871,0.000194450729921124,0.000226303009090751,0.000242229148675564,
0.000258155288260378,0.000258291104876511,0.000327654633620538,0.000399363990847956,
0.000469709285209015,0.000516310576520756),.UNSPECIFIED.);
#4820=B_SPLINE_CURVE_WITH_KNOTS('',3,(#214520,#214521,#214522,#214523,#214524,
#214525,#214526,#214527,#214528,#214529,#214530,#214531,#214532,#214533,
#214534,#214535,#214536,#214537,#214538,#214539,#214540,#214541,#214542,
#214543,#214544,#214545,#214546,#214547,#214548,#214549,#214550,#214551,
#214552,#214553,#214554,#214555,#214556,#214557,#214558,#214559),
 .UNSPECIFIED.,.F.,.F.,(4,3,3,3,3,3,3,3,3,3,3,3,3,4),(0.,6.84564250772788E-5,
0.00013828840658568,0.00020540747891715,0.000256966021225849,0.000257101146970263,
0.000271589374668166,0.000352213067611876,0.000388398097499787,0.000404123622054879,
0.000459162957997702,0.000486682625969114,0.00050044245995482,0.000514202293940525),
 .UNSPECIFIED.);
#4821=B_SPLINE_CURVE_WITH_KNOTS('',3,(#214563,#214564,#214565,#214566,#214567,
#214568,#214569,#214570,#214571,#214572,#214573,#214574,#214575,#214576,
#214577,#214578,#214579,#214580,#214581,#214582,#214583,#214584,#214585,
#214586,#214587,#214588,#214589,#214590,#214591,#214592,#214593,#214594,
#214595,#214596,#214597,#214598,#214599,#214600,#214601,#214602,#214603,
#214604,#214605),.UNSPECIFIED.,.F.,.F.,(4,3,3,3,3,3,3,3,3,3,3,3,3,3,4),
(1.73472347597681E-18,1.1289069806587E-5,7.65259666978257E-5,0.000102837507928504,
0.000112544869199246,0.000130746171581887,0.00019445072992113,0.000226303009090752,
0.000242229148675562,0.000258155288260373,0.000258291104876518,0.00032765463361364,
0.000399363990833812,0.000469709285188545,0.000516310576520745),
 .UNSPECIFIED.);
#4822=B_SPLINE_CURVE_WITH_KNOTS('',3,(#214613,#214614,#214615,#214616,#214617,
#214618,#214619,#214620,#214621,#214622,#214623,#214624,#214625,#214626,
#214627,#214628,#214629,#214630,#214631,#214632,#214633,#214634,#214635,
#214636,#214637,#214638,#214639,#214640,#214641,#214642,#214643,#214644,
#214645,#214646,#214647,#214648,#214649,#214650,#214651,#214652),
 .UNSPECIFIED.,.F.,.F.,(4,3,3,3,3,3,3,3,3,3,3,3,3,4),(0.,6.845642508068E-5,
0.000138288406592413,0.000205407478926651,0.000256966021225851,0.000257101146970266,
0.000271589374668168,0.000352213067602528,0.000388398097499775,0.000404123622054869,
0.0004591629579977,0.000486682625969116,0.000500442459954824,0.000514202293940531),
 .UNSPECIFIED.);
#4823=B_SPLINE_CURVE_WITH_KNOTS('',3,(#214656,#214657,#214658,#214659,#214660,
#214661,#214662,#214663,#214664,#214665,#214666,#214667,#214668,#214669,
#214670,#214671,#214672,#214673,#214674,#214675,#214676,#214677,#214678,
#214679,#214680,#214681,#214682,#214683,#214684,#214685,#214686,#214687,
#214688,#214689,#214690,#214691,#214692,#214693,#214694,#214695,#214696,
#214697,#214698),.UNSPECIFIED.,.F.,.F.,(4,3,3,3,3,3,3,3,3,3,3,3,3,3,4),
(0.,1.12890698065804E-5,7.65259667068095E-5,0.000102837507928478,0.000112544869199221,
0.000130746171581864,0.000194450729921116,0.000226303009090741,0.000242229148675554,
0.000258155288260367,0.000258291104876496,0.000327654633604266,0.00039936399081459,
0.000469709285160263,0.000516310576520733),.UNSPECIFIED.);
#4824=B_SPLINE_CURVE_WITH_KNOTS('',3,(#214705,#214706,#214707,#214708,#214709,
#214710,#214711,#214712,#214713,#214714,#214715,#214716,#214717,#214718,
#214719,#214720,#214721,#214722,#214723,#214724,#214725,#214726,#214727,
#214728,#214729,#214730,#214731,#214732,#214733,#214734,#214735,#214736,
#214737,#214738,#214739,#214740,#214741,#214742,#214743,#214744),
 .UNSPECIFIED.,.F.,.F.,(4,3,3,3,3,3,3,3,3,3,3,3,3,4),(0.,6.84564250814195E-5,
0.000138288406593869,0.000205407478929251,0.000256966021225844,0.000257101146970262,
0.000271589374668161,0.000352213067594447,0.000388398097499754,0.00040412362205485,
0.000459162957997688,0.000486682625969106,0.000500442459954816,0.000514202293940525),
 .UNSPECIFIED.);
#4825=B_SPLINE_CURVE_WITH_KNOTS('',3,(#214746,#214747,#214748,#214749,#214750,
#214751,#214752,#214753,#214754,#214755,#214756,#214757,#214758,#214759,
#214760,#214761,#214762,#214763,#214764,#214765,#214766,#214767,#214768,
#214769,#214770,#214771,#214772,#214773,#214774,#214775,#214776,#214777,
#214778,#214779,#214780,#214781,#214782,#214783,#214784,#214785,#214786,
#214787,#214788),.UNSPECIFIED.,.F.,.F.,(4,3,3,3,3,3,3,3,3,3,3,3,3,3,4),
(0.,1.12890698065878E-5,7.65259667079882E-5,0.000102837507928575,0.000112544869199312,
0.000130746171581944,0.000194450729921155,0.000226303009090761,0.000242229148675564,
0.000258155288260367,0.000258291104876521,0.00032765463362058,0.000399363990847816,
0.000469709285208397,0.000516310576520733),.UNSPECIFIED.);
#4826=B_SPLINE_CURVE_WITH_KNOTS('',3,(#214796,#214797,#214798,#214799,#214800,
#214801,#214802,#214803,#214804,#214805,#214806,#214807,#214808,#214809,
#214810,#214811,#214812,#214813,#214814,#214815,#214816,#214817,#214818,
#214819,#214820,#214821,#214822,#214823,#214824,#214825,#214826,#214827,
#214828,#214829,#214830,#214831,#214832,#214833,#214834,#214835),
 .UNSPECIFIED.,.F.,.F.,(4,3,3,3,3,3,3,3,3,3,3,3,3,4),(0.,6.84564250828593E-5,
0.000138288406596549,0.000205407478932344,0.000256966021225844,0.000257101146970264,
0.00027158937466816,0.000352213067602491,0.000388398097499745,0.000404123622054843,
0.000459162957997685,0.000486682625969106,0.000500442459954816,0.000514202293940527),
 .UNSPECIFIED.);
#4827=B_SPLINE_CURVE_WITH_KNOTS('',3,(#214839,#214840,#214841,#214842,#214843,
#214844,#214845,#214846,#214847,#214848,#214849,#214850,#214851,#214852,
#214853,#214854,#214855,#214856,#214857,#214858,#214859,#214860,#214861,
#214862,#214863,#214864,#214865,#214866,#214867,#214868,#214869,#214870,
#214871,#214872,#214873,#214874,#214875,#214876,#214877,#214878,#214879,
#214880,#214881),.UNSPECIFIED.,.F.,.F.,(4,3,3,3,3,3,3,3,3,3,3,3,3,3,4),
(0.,1.12890698065845E-5,7.65259667089463E-5,0.000102837507928522,0.000112544869199262,
0.0001307461715819,0.000194450729921135,0.000226303009090752,0.000242229148675561,
0.000258155288260369,0.000258291104876517,0.000327654633616968,0.000399363990840608,
0.00046970928519815,0.000516310576520738),.UNSPECIFIED.);
#4828=B_SPLINE_CURVE_WITH_KNOTS('',3,(#214889,#214890,#214891,#214892,#214893,
#214894,#214895,#214896,#214897,#214898,#214899,#214900,#214901,#214902,
#214903,#214904,#214905,#214906,#214907,#214908,#214909,#214910,#214911,
#214912,#214913,#214914,#214915,#214916,#214917,#214918,#214919,#214920,
#214921,#214922,#214923,#214924,#214925,#214926,#214927,#214928),
 .UNSPECIFIED.,.F.,.F.,(4,3,3,3,3,3,3,3,3,3,3,3,3,4),(4.33680868994202E-19,
6.8456425081903E-5,0.000138288406594929,0.000205407478930537,0.000256966021225847,
0.000257101146970261,0.000271589374668165,0.000352213067606131,0.000388398097499846,
0.00040412362205493,0.000459162957997726,0.000486682625969123,0.000500442459954822,
0.000514202293940521),.UNSPECIFIED.);
#4829=B_SPLINE_CURVE_WITH_KNOTS('',3,(#214932,#214933,#214934,#214935,#214936,
#214937,#214938,#214939,#214940,#214941,#214942,#214943,#214944,#214945,
#214946,#214947,#214948,#214949,#214950,#214951,#214952,#214953,#214954,
#214955,#214956,#214957,#214958,#214959,#214960,#214961,#214962,#214963,
#214964,#214965,#214966,#214967,#214968,#214969,#214970,#214971,#214972,
#214973,#214974),.UNSPECIFIED.,.F.,.F.,(4,3,3,3,3,3,3,3,3,3,3,3,3,3,4),
(0.,1.12890698065809E-5,7.65259667023175E-5,0.000102837507928505,0.000112544869199247,
0.000130746171581888,0.000194450729921132,0.000226303009090755,0.000242229148675566,
0.000258155288260377,0.000258291104876515,0.000327654633619138,0.000399363990844944,
0.000469709285204301,0.000516310576520754),.UNSPECIFIED.);
#4830=B_SPLINE_CURVE_WITH_KNOTS('',3,(#214982,#214983,#214984,#214985,#214986,
#214987,#214988,#214989,#214990,#214991,#214992,#214993,#214994,#214995,
#214996,#214997,#214998,#214999,#215000,#215001,#215002,#215003,#215004,
#215005,#215006,#215007,#215008,#215009,#215010,#215011,#215012,#215013,
#215014,#215015,#215016,#215017,#215018,#215019,#215020,#215021),
 .UNSPECIFIED.,.F.,.F.,(4,3,3,3,3,3,3,3,3,3,3,3,3,4),(0.,6.84564250785299E-5,
0.00013828840658849,0.000205407478922068,0.000256966021225852,0.00025710114697026,
0.000271589374668164,0.000352213067604385,0.000388398097499773,0.000404123622054867,
0.000459162957997693,0.000486682625969106,0.000500442459954813,0.000514202293940519),
 .UNSPECIFIED.);
#4831=B_SPLINE_CURVE_WITH_KNOTS('',3,(#215025,#215026,#215027,#215028,#215029,
#215030,#215031,#215032,#215033,#215034,#215035,#215036,#215037,#215038,
#215039,#215040,#215041,#215042,#215043,#215044,#215045,#215046,#215047,
#215048,#215049,#215050,#215051,#215052,#215053,#215054,#215055,#215056,
#215057,#215058,#215059,#215060,#215061,#215062,#215063,#215064,#215065,
#215066,#215067),.UNSPECIFIED.,.F.,.F.,(4,3,3,3,3,3,3,3,3,3,3,3,3,3,4),
(0.,1.12890698065803E-5,7.65259667084363E-5,0.00010283750792847,0.000112544869199214,
0.000130746171581859,0.000194450729921117,0.000226303009090746,0.000242229148675561,
0.000258155288260375,0.000258291104876523,0.000327654633608061,0.000399363990822207,
0.000469709285171161,0.00051631057652075),.UNSPECIFIED.);
#4832=B_SPLINE_CURVE_WITH_KNOTS('',3,(#215075,#215076,#215077,#215078,#215079,
#215080,#215081,#215082,#215083,#215084,#215085,#215086,#215087,#215088,
#215089,#215090,#215091,#215092,#215093,#215094,#215095,#215096,#215097,
#215098,#215099,#215100,#215101,#215102,#215103,#215104,#215105,#215106,
#215107,#215108,#215109,#215110,#215111,#215112,#215113,#215114),
 .UNSPECIFIED.,.F.,.F.,(4,3,3,3,3,3,3,3,3,3,3,3,3,4),(2.16840434497101E-18,
6.84564250825956E-5,0.000138288406596379,0.000205407478932536,0.000256966021225845,
0.000257101146970259,0.000271589374668164,0.000352213067616007,0.000388398097499831,
0.000404123622054917,0.000459162957997717,0.000486682625969117,0.000500442459954816,
0.000514202293940516),.UNSPECIFIED.);
#4833=B_SPLINE_CURVE_WITH_KNOTS('',3,(#215118,#215119,#215120,#215121,#215122,
#215123,#215124,#215125,#215126,#215127,#215128,#215129,#215130,#215131,
#215132,#215133,#215134,#215135,#215136,#215137,#215138,#215139,#215140,
#215141,#215142,#215143,#215144,#215145,#215146,#215147,#215148,#215149,
#215150,#215151,#215152,#215153,#215154,#215155,#215156,#215157,#215158,
#215159,#215160),.UNSPECIFIED.,.F.,.F.,(4,3,3,3,3,3,3,3,3,3,3,3,3,3,4),
(0.,1.12890698065779E-5,7.6525966700619E-5,0.000102837507928493,0.000112544869199235,
0.000130746171581877,0.000194450729921122,0.000226303009090745,0.000242229148675556,
0.000258155288260368,0.000258291104876509,0.000327654633624863,0.000399363990856454,
0.000469709285220816,0.000516310576520735),.UNSPECIFIED.);
#4834=B_SPLINE_CURVE_WITH_KNOTS('',3,(#215168,#215169,#215170,#215171,#215172,
#215173,#215174,#215175,#215176,#215177,#215178,#215179,#215180,#215181,
#215182,#215183,#215184,#215185,#215186,#215187,#215188,#215189,#215190,
#215191,#215192,#215193,#215194,#215195,#215196,#215197,#215198,#215199,
#215200,#215201,#215202,#215203,#215204,#215205,#215206,#215207),
 .UNSPECIFIED.,.F.,.F.,(4,3,3,3,3,3,3,3,3,3,3,3,3,4),(0.,6.84564250783218E-5,
0.000138288406587982,0.000205407478921425,0.000256966021225847,0.000257101146970263,
0.000271589374668172,0.000352213067602529,0.000388398097499895,0.000404123622054973,
0.000459162957997745,0.000486682625969131,0.000500442459954824,0.000514202293940517),
 .UNSPECIFIED.);
#4835=B_SPLINE_CURVE_WITH_KNOTS('',3,(#215211,#215212,#215213,#215214,#215215,
#215216,#215217,#215218,#215219,#215220,#215221,#215222,#215223,#215224,
#215225,#215226,#215227,#215228,#215229,#215230,#215231,#215232,#215233,
#215234,#215235,#215236,#215237,#215238,#215239,#215240,#215241,#215242,
#215243,#215244,#215245,#215246,#215247,#215248,#215249,#215250,#215251,
#215252,#215253),.UNSPECIFIED.,.F.,.F.,(4,3,3,3,3,3,3,3,3,3,3,3,3,3,4),
(0.,1.12890698065829E-5,7.6525966723226E-5,0.000102837507928496,0.000112544869199238,
0.00013074617158188,0.000194450729921127,0.000226303009090751,0.000242229148675563,
0.000258155288260374,0.000258291104876528,0.000327654633609462,0.000399363990825717,
0.000469709285176748,0.000516310576520749),.UNSPECIFIED.);
#4836=B_SPLINE_CURVE_WITH_KNOTS('',3,(#215261,#215262,#215263,#215264,#215265,
#215266,#215267,#215268,#215269,#215270,#215271,#215272,#215273,#215274,
#215275,#215276,#215277,#215278,#215279,#215280,#215281,#215282,#215283,
#215284,#215285,#215286,#215287,#215288,#215289,#215290,#215291,#215292,
#215293,#215294,#215295,#215296,#215297,#215298,#215299,#215300),
 .UNSPECIFIED.,.F.,.F.,(4,3,3,3,3,3,3,3,3,3,3,3,3,4),(2.60208521396521E-18,
6.84564250868235E-5,0.000138288406605512,0.00020540747894714,0.000256966021225843,
0.00025710114697026,0.000271589374668176,0.000352213067624583,0.000388398097499925,
0.000404123622054999,0.000459162957997759,0.000486682625969138,0.000500442459954828,
0.000514202293940518),.UNSPECIFIED.);
#4837=B_SPLINE_CURVE_WITH_KNOTS('',3,(#215304,#215305,#215306,#215307,#215308,
#215309,#215310,#215311,#215312,#215313,#215314,#215315,#215316,#215317,
#215318,#215319,#215320,#215321,#215322,#215323,#215324,#215325,#215326,
#215327,#215328,#215329,#215330,#215331,#215332,#215333,#215334,#215335,
#215336,#215337,#215338,#215339,#215340,#215341,#215342,#215343,#215344,
#215345,#215346),.UNSPECIFIED.,.F.,.F.,(4,3,3,3,3,3,3,3,3,3,3,3,3,3,4),
(0.,1.12890698065793E-5,7.65259667123674E-5,0.000102837507928489,0.000112544869199231,
0.000130746171581874,0.000194450729921124,0.000226303009090748,0.000242229148675561,
0.000258155288260373,0.000258291104876523,0.000327654633615003,0.000399363990836477,
0.000469709285191897,0.000516310576520746),.UNSPECIFIED.);
#4838=B_SPLINE_CURVE_WITH_KNOTS('',3,(#215354,#215355,#215356,#215357,#215358,
#215359,#215360,#215361,#215362,#215363,#215364,#215365,#215366,#215367,
#215368,#215369,#215370,#215371,#215372,#215373,#215374,#215375,#215376,
#215377,#215378,#215379,#215380,#215381,#215382,#215383,#215384,#215385,
#215386,#215387,#215388,#215389,#215390,#215391,#215392,#215393),
 .UNSPECIFIED.,.F.,.F.,(4,3,3,3,3,3,3,3,3,3,3,3,3,4),(1.73472347597681E-18,
6.845642508305E-5,0.000138288406596686,0.000205407478931409,0.000256966021225855,
0.000257101146970272,0.000271589374668164,0.000352213067614368,0.000388398097499747,
0.000404123622054847,0.000459162957997695,0.000486682625969118,0.00050044245995483,
0.000514202293940542),.UNSPECIFIED.);
#4839=B_SPLINE_CURVE_WITH_KNOTS('',3,(#215397,#215398,#215399,#215400,#215401,
#215402,#215403,#215404,#215405,#215406,#215407,#215408,#215409,#215410,
#215411,#215412,#215413,#215414,#215415,#215416,#215417,#215418,#215419,
#215420,#215421,#215422,#215423,#215424,#215425,#215426,#215427,#215428,
#215429,#215430,#215431,#215432,#215433,#215434,#215435,#215436,#215437,
#215438,#215439),.UNSPECIFIED.,.F.,.F.,(4,3,3,3,3,3,3,3,3,3,3,3,3,3,4),
(0.,1.12890698065779E-5,7.65259666775026E-5,0.00010283750792847,0.000112544869199214,
0.000130746171581858,0.000194450729921113,0.000226303009090741,0.000242229148675555,
0.000258155288260369,0.00025829110487651,0.000327654633629564,0.000399363990865801,
0.000469709285235127,0.000516310576520737),.UNSPECIFIED.);
#4840=B_SPLINE_CURVE_WITH_KNOTS('',3,(#215447,#215448,#215449,#215450,#215451,
#215452,#215453,#215454,#215455,#215456,#215457,#215458,#215459,#215460,
#215461,#215462,#215463,#215464,#215465,#215466,#215467,#215468,#215469,
#215470,#215471,#215472,#215473,#215474,#215475,#215476,#215477,#215478,
#215479,#215480,#215481,#215482,#215483,#215484,#215485,#215486),
 .UNSPECIFIED.,.F.,.F.,(4,3,3,3,3,3,3,3,3,3,3,3,3,4),(0.,6.84564250806006E-5,
0.000138288406591434,0.000205407478922972,0.000256966021225842,0.000257101146970266,
0.000271589374668167,0.000352213067618348,0.000388398097499851,0.000404123622054936,
0.000459162957997734,0.000486682625969134,0.000500442459954833,0.000514202293940533),
 .UNSPECIFIED.);
#4841=B_SPLINE_CURVE_WITH_KNOTS('',3,(#215490,#215491,#215492,#215493,#215494,
#215495,#215496,#215497,#215498,#215499,#215500,#215501,#215502,#215503,
#215504,#215505,#215506,#215507,#215508,#215509,#215510,#215511,#215512,
#215513,#215514,#215515,#215516,#215517,#215518,#215519,#215520,#215521,
#215522,#215523,#215524,#215525,#215526,#215527,#215528,#215529,#215530,
#215531,#215532),.UNSPECIFIED.,.F.,.F.,(4,3,3,3,3,3,3,3,3,3,3,3,3,3,4),
(0.,1.12890698065802E-5,7.6525966703759E-5,0.000102837507928505,0.000112544869199247,
0.000130746171581888,0.000194450729921132,0.000226303009090754,0.000242229148675565,
0.000258155288260376,0.000258291104876512,0.000327654633617546,0.000399363990841935,
0.00046970928520053,0.000516310576520752),.UNSPECIFIED.);
#4842=B_SPLINE_CURVE_WITH_KNOTS('',3,(#215540,#215541,#215542,#215543,#215544,
#215545,#215546,#215547,#215548,#215549,#215550,#215551,#215552,#215553,
#215554,#215555,#215556,#215557,#215558,#215559,#215560,#215561,#215562,
#215563,#215564,#215565,#215566,#215567,#215568,#215569,#215570,#215571,
#215572,#215573,#215574,#215575,#215576,#215577,#215578,#215579),
 .UNSPECIFIED.,.F.,.F.,(4,3,3,3,3,3,3,3,3,3,3,3,3,4),(0.,6.84564250876636E-5,
0.000138288406606712,0.000205407478948682,0.000256966021225854,0.000257101146970261,
0.00027158937466816,0.000352213067590487,0.000388398097499747,0.000404123622054844,
0.000459162957997683,0.000486682625969103,0.000500442459954813,0.000514202293940522),
 .UNSPECIFIED.);
#4843=B_SPLINE_CURVE_WITH_KNOTS('',3,(#215583,#215584,#215585,#215586,#215587,
#215588,#215589,#215590,#215591,#215592,#215593,#215594,#215595,#215596,
#215597,#215598,#215599,#215600,#215601,#215602,#215603,#215604,#215605,
#215606,#215607,#215608,#215609,#215610,#215611,#215612,#215613,#215614,
#215615,#215616,#215617,#215618,#215619,#215620,#215621,#215622,#215623,
#215624,#215625),.UNSPECIFIED.,.F.,.F.,(4,3,3,3,3,3,3,3,3,3,3,3,3,3,4),
(0.,1.12890698065826E-5,7.65259666897135E-5,0.000102837507928503,0.000112544869199245,
0.000130746171581886,0.00019445072992113,0.000226303009090752,0.000242229148675564,
0.000258155288260375,0.00025829110487651,0.000327654633619508,0.000399363990844196,
0.000469709285200996,0.000516310576520749),.UNSPECIFIED.);
#4844=B_SPLINE_CURVE_WITH_KNOTS('',3,(#215633,#215634,#215635,#215636,#215637,
#215638,#215639,#215640,#215641,#215642,#215643,#215644,#215645,#215646,
#215647,#215648,#215649,#215650,#215651,#215652,#215653,#215654,#215655,
#215656,#215657,#215658,#215659,#215660,#215661,#215662,#215663,#215664,
#215665,#215666,#215667,#215668,#215669,#215670,#215671,#215672),
 .UNSPECIFIED.,.F.,.F.,(4,3,3,3,3,3,3,3,3,3,3,3,3,4),(2.60208521396521E-18,
6.84564250877193E-5,0.000138288406606367,0.000205407478946553,0.000256966021225849,
0.000257101146970267,0.000271589374668177,0.000352213067599024,0.000388398097499851,
0.000404123622054936,0.000459162957997734,0.000486682625969133,0.000500442459954832,
0.000514202293940532),.UNSPECIFIED.);
#4845=B_SPLINE_CURVE_WITH_KNOTS('',3,(#215676,#215677,#215678,#215679,#215680,
#215681,#215682,#215683,#215684,#215685,#215686,#215687,#215688,#215689,
#215690,#215691,#215692,#215693,#215694,#215695,#215696,#215697,#215698,
#215699,#215700,#215701,#215702,#215703,#215704,#215705,#215706,#215707,
#215708,#215709,#215710,#215711,#215712,#215713,#215714,#215715,#215716,
#215717,#215718),.UNSPECIFIED.,.F.,.F.,(4,3,3,3,3,3,3,3,3,3,3,3,3,3,4),
(0.,1.12890698065771E-5,7.65259667020667E-5,0.000102837507928448,0.000112544869199193,
0.00013074617158184,0.000194450729921102,0.000226303009090734,0.000242229148675549,
0.000258155288260365,0.000258291104876513,0.000327654633616971,0.000399363990840478,
0.000469709285197867,0.000516310576520737),.UNSPECIFIED.);
#4846=B_SPLINE_CURVE_WITH_KNOTS('',3,(#215726,#215727,#215728,#215729,#215730,
#215731,#215732,#215733,#215734,#215735,#215736,#215737,#215738,#215739,
#215740,#215741,#215742,#215743,#215744,#215745,#215746,#215747,#215748,
#215749,#215750,#215751,#215752,#215753,#215754,#215755,#215756,#215757,
#215758,#215759,#215760,#215761,#215762,#215763,#215764,#215765),
 .UNSPECIFIED.,.F.,.F.,(4,3,3,3,3,3,3,3,3,3,3,3,3,4),(0.,6.84564250802978E-5,
0.000138288406591518,0.000205407478925098,0.000256966021225857,0.000257101146970261,
0.000271589374668162,0.000352213067612065,0.000388398097499789,0.000404123622054881,
0.000459162957997701,0.000486682625969112,0.000500442459954817,0.000514202293940522),
 .UNSPECIFIED.);
#4847=B_SPLINE_CURVE_WITH_KNOTS('',3,(#215769,#215770,#215771,#215772,#215773,
#215774,#215775,#215776,#215777,#215778,#215779,#215780,#215781,#215782,
#215783,#215784,#215785,#215786,#215787,#215788,#215789,#215790,#215791,
#215792,#215793,#215794,#215795,#215796,#215797,#215798,#215799,#215800,
#215801,#215802,#215803,#215804,#215805,#215806,#215807,#215808,#215809,
#215810,#215811),.UNSPECIFIED.,.F.,.F.,(4,3,3,3,3,3,3,3,3,3,3,3,3,3,4),
(0.,1.12890698065831E-5,7.65259667143359E-5,0.000102837507928517,0.000112544869199258,
0.000130746171581897,0.000194450729921133,0.000226303009090751,0.00024222914867556,
0.000258155288260369,0.000258291104876512,0.000327654633615957,0.000399363990839121,
0.000469709285196728,0.000516310576520738),.UNSPECIFIED.);
#4848=B_SPLINE_CURVE_WITH_KNOTS('',3,(#215819,#215820,#215821,#215822,#215823,
#215824,#215825,#215826,#215827,#215828,#215829,#215830,#215831,#215832,
#215833,#215834,#215835,#215836,#215837,#215838,#215839,#215840,#215841,
#215842,#215843,#215844,#215845,#215846,#215847,#215848,#215849,#215850,
#215851,#215852,#215853,#215854,#215855,#215856,#215857,#215858),
 .UNSPECIFIED.,.F.,.F.,(4,3,3,3,3,3,3,3,3,3,3,3,3,4),(0.,6.8456425084354E-5,
0.000138288406599791,0.000205407478937876,0.000256966021225842,0.000257101146970262,
0.000271589374668162,0.000352213067600001,0.00038839809749976,0.000404123622054856,
0.00045916295799769,0.000486682625969107,0.000500442459954816,0.000514202293940525),
 .UNSPECIFIED.);
#4849=B_SPLINE_CURVE_WITH_KNOTS('',3,(#215862,#215863,#215864,#215865,#215866,
#215867,#215868,#215869,#215870,#215871,#215872,#215873,#215874,#215875,
#215876,#215877,#215878,#215879,#215880,#215881,#215882,#215883,#215884,
#215885,#215886,#215887,#215888,#215889,#215890,#215891,#215892,#215893,
#215894,#215895,#215896,#215897,#215898,#215899,#215900,#215901,#215902,
#215903,#215904),.UNSPECIFIED.,.F.,.F.,(4,3,3,3,3,3,3,3,3,3,3,3,3,3,4),
(0.,1.12890698065845E-5,7.65259667118142E-5,0.000102837507928515,0.000112544869199256,
0.000130746171581896,0.000194450729921136,0.000226303009090755,0.000242229148675565,
0.000258155288260375,0.000258291104876512,0.000327654633609095,0.000399363990824695,
0.000469709285175208,0.00051631057652075),.UNSPECIFIED.);
#4850=B_SPLINE_CURVE_WITH_KNOTS('',3,(#215912,#215913,#215914,#215915,#215916,
#215917,#215918,#215919,#215920,#215921,#215922,#215923,#215924,#215925,
#215926,#215927,#215928,#215929,#215930,#215931,#215932,#215933,#215934,
#215935,#215936,#215937,#215938,#215939,#215940,#215941,#215942,#215943,
#215944,#215945,#215946,#215947,#215948,#215949,#215950,#215951),
 .UNSPECIFIED.,.F.,.F.,(4,3,3,3,3,3,3,3,3,3,3,3,3,4),(0.,6.84564250776835E-5,
0.000138288406586343,0.000205407478917895,0.000256966021225848,0.000257101146970261,
0.000271589374668164,0.000352213067606,0.000388398097499787,0.000404123622054879,
0.0004591629579977,0.000486682625969111,0.000500442459954816,0.000514202293940522),
 .UNSPECIFIED.);
#4851=B_SPLINE_CURVE_WITH_KNOTS('',3,(#215955,#215956,#215957,#215958,#215959,
#215960,#215961,#215962,#215963,#215964,#215965,#215966,#215967,#215968,
#215969,#215970,#215971,#215972,#215973,#215974,#215975,#215976,#215977,
#215978,#215979,#215980,#215981,#215982,#215983,#215984,#215985,#215986,
#215987,#215988,#215989,#215990,#215991,#215992,#215993,#215994,#215995,
#215996,#215997),.UNSPECIFIED.,.F.,.F.,(4,3,3,3,3,3,3,3,3,3,3,3,3,3,4),
(1.73472347597681E-18,1.12890698065845E-5,7.65259667057065E-5,0.000102837507928531,
0.000112544869199271,0.000130746171581908,0.000194450729921137,0.000226303009090752,
0.00024222914867556,0.000258155288260367,0.000258291104876518,0.000327654633610688,
0.000399363990827742,0.000469709285179423,0.000516310576520732),
 .UNSPECIFIED.);
#4852=B_SPLINE_CURVE_WITH_KNOTS('',3,(#216005,#216006,#216007,#216008,#216009,
#216010,#216011,#216012,#216013,#216014,#216015,#216016,#216017,#216018,
#216019,#216020,#216021,#216022,#216023,#216024,#216025,#216026,#216027,
#216028,#216029,#216030,#216031,#216032,#216033,#216034,#216035,#216036,
#216037,#216038,#216039,#216040,#216041,#216042,#216043,#216044),
 .UNSPECIFIED.,.F.,.F.,(4,3,3,3,3,3,3,3,3,3,3,3,3,4),(0.,6.84564250845372E-5,
0.000138288406600476,0.000205407478939388,0.000256966021225852,0.000257101146970261,
0.000271589374668165,0.000352213067598438,0.000388398097499816,0.000404123622054904,
0.000459162957997713,0.000486682625969117,0.000500442459954819,0.000514202293940521),
 .UNSPECIFIED.);
#4853=B_SPLINE_CURVE_WITH_KNOTS('',3,(#216048,#216049,#216050,#216051,#216052,
#216053,#216054,#216055,#216056,#216057,#216058,#216059,#216060,#216061,
#216062,#216063,#216064,#216065,#216066,#216067,#216068,#216069,#216070,
#216071,#216072,#216073,#216074,#216075,#216076,#216077,#216078,#216079,
#216080,#216081,#216082,#216083,#216084,#216085,#216086,#216087,#216088,
#216089,#216090),.UNSPECIFIED.,.F.,.F.,(4,3,3,3,3,3,3,3,3,3,3,3,3,3,4),
(8.67361737988403E-19,1.12890698065789E-5,7.65259667078676E-5,0.000102837507928473,
0.000112544869199216,0.00013074617158186,0.000194450729921113,0.000226303009090739,
0.000242229148675552,0.000258155288260366,0.000258291104876509,0.000327654633616604,
0.000399363990839486,0.000469709285196016,0.00051631057652073),
 .UNSPECIFIED.);
#4854=B_SPLINE_CURVE_WITH_KNOTS('',3,(#216097,#216098,#216099,#216100,#216101,
#216102,#216103,#216104,#216105,#216106,#216107,#216108,#216109,#216110,
#216111,#216112,#216113,#216114,#216115,#216116,#216117,#216118,#216119,
#216120,#216121,#216122,#216123,#216124,#216125,#216126,#216127,#216128,
#216129,#216130,#216131,#216132,#216133,#216134,#216135,#216136),
 .UNSPECIFIED.,.F.,.F.,(4,3,3,3,3,3,3,3,3,3,3,3,3,4),(0.,6.8456425078443E-5,
0.000138288406587804,0.000205407478920017,0.000256966021225852,0.000257101146970261,
0.000271589374668165,0.000352213067601245,0.000388398097499795,0.000404123622054885,
0.000459162957997703,0.000486682625969112,0.000500442459954817,0.000514202293940521),
 .UNSPECIFIED.);
#4855=B_SPLINE_CURVE_WITH_KNOTS('',3,(#216139,#216140,#216141,#216142,#216143,
#216144,#216145,#216146,#216147,#216148,#216149,#216150,#216151,#216152,
#216153,#216154,#216155,#216156,#216157,#216158,#216159,#216160,#216161,
#216162,#216163,#216164,#216165,#216166,#216167,#216168,#216169,#216170,
#216171,#216172,#216173,#216174,#216175),.UNSPECIFIED.,.F.,.F.,(4,3,3,3,
3,3,3,3,3,3,3,3,4),(0.,1.12535551670991E-5,7.76936938516679E-5,0.000102513517961096,
0.000121879189824247,0.000189659041345274,0.000223548967105788,0.000257294099096098,
0.000257438892866301,0.00032572085175526,0.000396486773955018,0.00046624270766206,
0.000514877785732602),.UNSPECIFIED.);
#4856=B_SPLINE_CURVE_WITH_KNOTS('',3,(#216183,#216184,#216185,#216186,#216187,
#216188,#216189,#216190,#216191,#216192,#216193,#216194,#216195,#216196,
#216197,#216198,#216199,#216200,#216201,#216202,#216203,#216204,#216205,
#216206,#216207,#216208,#216209,#216210,#216211,#216212,#216213,#216214,
#216215,#216216,#216217,#216218,#216219,#216220,#216221,#216222),
 .UNSPECIFIED.,.F.,.F.,(4,3,3,3,3,3,3,3,3,3,3,3,3,4),(0.,6.80370855387726E-5,
0.00013730316930294,0.000203636706669859,0.000256396220959708,0.000256540237295739,
0.000285209320207746,0.000342105100635664,0.000384776935956602,0.000400778874201954,
0.000456785658060685,0.000484789049990051,0.000498790745954733,0.000512792441919416),
 .UNSPECIFIED.);
#4857=B_SPLINE_CURVE_WITH_KNOTS('',3,(#216226,#216227,#216228,#216229,#216230,
#216231,#216232,#216233,#216234,#216235,#216236,#216237,#216238,#216239,
#216240,#216241,#216242,#216243,#216244,#216245,#216246,#216247,#216248,
#216249,#216250,#216251,#216252,#216253,#216254,#216255,#216256,#216257,
#216258,#216259,#216260,#216261,#216262),.UNSPECIFIED.,.F.,.F.,(4,3,3,3,
3,3,3,3,3,3,3,3,4),(0.,1.12535551670995E-5,7.76936938481029E-5,0.000102513517961135,
0.00012187918982428,0.000189659041345289,0.000223548967105794,0.000257294099096101,
0.000257438892866298,0.000325720851760917,0.000396486773966304,0.000466242707678062,
0.000514877785732596),.UNSPECIFIED.);
#4858=B_SPLINE_CURVE_WITH_KNOTS('',3,(#216270,#216271,#216272,#216273,#216274,
#216275,#216276,#216277,#216278,#216279,#216280,#216281,#216282,#216283,
#216284,#216285,#216286,#216287,#216288,#216289,#216290,#216291,#216292,
#216293,#216294,#216295,#216296,#216297,#216298,#216299,#216300,#216301,
#216302,#216303,#216304,#216305,#216306,#216307,#216308,#216309),
 .UNSPECIFIED.,.F.,.F.,(4,3,3,3,3,3,3,3,3,3,3,3,3,4),(0.,6.80370855360972E-5,
0.000137303169297683,0.000203636706662521,0.000256396220959706,0.000256540237295735,
0.00028520932020774,0.000342105100635658,0.000384776935956597,0.000400778874201949,
0.00045678565806068,0.000484789049990046,0.000498790745954729,0.000512792441919412),
 .UNSPECIFIED.);
#4859=B_SPLINE_CURVE_WITH_KNOTS('',3,(#216313,#216314,#216315,#216316,#216317,
#216318,#216319,#216320,#216321,#216322,#216323,#216324,#216325,#216326,
#216327,#216328,#216329,#216330,#216331,#216332,#216333,#216334,#216335,
#216336,#216337,#216338,#216339,#216340,#216341,#216342,#216343,#216344,
#216345,#216346,#216347,#216348,#216349),.UNSPECIFIED.,.F.,.F.,(4,3,3,3,
3,3,3,3,3,3,3,3,4),(0.,1.12535551671024E-5,7.76936938462203E-5,0.000102513517961152,
0.000121879189824295,0.000189659041345298,0.000223548967105799,0.000257294099096102,
0.000257438892866301,0.00032572085176373,0.00039648677397213,0.000466242707686686,
0.000514877785732602),.UNSPECIFIED.);
#4860=B_SPLINE_CURVE_WITH_KNOTS('',3,(#216357,#216358,#216359,#216360,#216361,
#216362,#216363,#216364,#216365,#216366,#216367,#216368,#216369,#216370,
#216371,#216372,#216373,#216374,#216375,#216376,#216377,#216378,#216379,
#216380,#216381,#216382,#216383,#216384,#216385,#216386,#216387,#216388,
#216389,#216390,#216391,#216392,#216393,#216394,#216395,#216396),
 .UNSPECIFIED.,.F.,.F.,(4,3,3,3,3,3,3,3,3,3,3,3,3,4),(0.,6.80370855362733E-5,
0.00013730316929717,0.000203636706659883,0.000256396220959707,0.000256540237295737,
0.000285209320207728,0.000342105100635649,0.000384776935956591,0.000400778874201944,
0.000456785658060679,0.000484789049990047,0.00049879074595473,0.000512792441919414),
 .UNSPECIFIED.);
#4861=B_SPLINE_CURVE_WITH_KNOTS('',3,(#216400,#216401,#216402,#216403,#216404,
#216405,#216406,#216407,#216408,#216409,#216410,#216411,#216412,#216413,
#216414,#216415,#216416,#216417,#216418,#216419,#216420,#216421,#216422,
#216423,#216424,#216425,#216426,#216427,#216428,#216429,#216430,#216431,
#216432,#216433,#216434,#216435,#216436),.UNSPECIFIED.,.F.,.F.,(4,3,3,3,
3,3,3,3,3,3,3,3,4),(0.,1.12535551670993E-5,7.7693693845788E-5,0.000102513517961118,
0.000121879189824266,0.000189659041345283,0.000223548967105792,0.000257294099096107,
0.000257438892866301,0.000325720851757369,0.000396486773959682,0.000466242707669865,
0.000514877785732601),.UNSPECIFIED.);
#4862=B_SPLINE_CURVE_WITH_KNOTS('',3,(#216444,#216445,#216446,#216447,#216448,
#216449,#216450,#216451,#216452,#216453,#216454,#216455,#216456,#216457,
#216458,#216459,#216460,#216461,#216462,#216463,#216464,#216465,#216466,
#216467,#216468,#216469,#216470,#216471,#216472,#216473,#216474,#216475,
#216476,#216477,#216478,#216479,#216480,#216481,#216482,#216483),
 .UNSPECIFIED.,.F.,.F.,(4,3,3,3,3,3,3,3,3,3,3,3,3,4),(0.,6.80370855408422E-5,
0.000137303169306678,0.000203636706674689,0.000256396220959706,0.000256540237295731,
0.000285209320207737,0.000342105100635656,0.000384776935956595,0.000400778874201947,
0.000456785658060679,0.000484789049990045,0.000498790745954728,0.000512792441919411),
 .UNSPECIFIED.);
#4863=B_SPLINE_CURVE_WITH_KNOTS('',3,(#216487,#216488,#216489,#216490,#216491,
#216492,#216493,#216494,#216495,#216496,#216497,#216498,#216499,#216500,
#216501,#216502,#216503,#216504,#216505,#216506,#216507,#216508,#216509,
#216510,#216511,#216512,#216513,#216514,#216515,#216516,#216517,#216518,
#216519,#216520,#216521,#216522,#216523),.UNSPECIFIED.,.F.,.F.,(4,3,3,3,
3,3,3,3,3,3,3,3,4),(0.,1.1253555167101E-5,7.76936938405201E-5,0.00010251351796113,
0.000121879189824277,0.000189659041345291,0.000223548967105797,0.000257294099096104,
0.000257438892866304,0.000325720851758851,0.000396486773962169,0.000466242707672447,
0.000514877785732608),.UNSPECIFIED.);
#4864=B_SPLINE_CURVE_WITH_KNOTS('',3,(#216531,#216532,#216533,#216534,#216535,
#216536,#216537,#216538,#216539,#216540,#216541,#216542,#216543,#216544,
#216545,#216546,#216547,#216548,#216549,#216550,#216551,#216552,#216553,
#216554,#216555,#216556,#216557,#216558,#216559,#216560,#216561,#216562,
#216563,#216564,#216565,#216566,#216567,#216568,#216569,#216570),
 .UNSPECIFIED.,.F.,.F.,(4,3,3,3,3,3,3,3,3,3,3,3,3,4),(0.,6.80370855415949E-5,
0.000137303169308611,0.000203636706678468,0.00025639622095971,0.000256540237295739,
0.000285209320207752,0.000342105100635669,0.000384776935956607,0.000400778874201959,
0.000456785658060689,0.000484789049990055,0.000498790745954737,0.00051279244191942),
 .UNSPECIFIED.);
#4865=B_SPLINE_CURVE_WITH_KNOTS('',3,(#216574,#216575,#216576,#216577,#216578,
#216579,#216580,#216581,#216582,#216583,#216584,#216585,#216586,#216587,
#216588,#216589,#216590,#216591,#216592,#216593,#216594,#216595,#216596,
#216597,#216598,#216599,#216600,#216601,#216602,#216603,#216604,#216605,
#216606,#216607,#216608,#216609,#216610),.UNSPECIFIED.,.F.,.F.,(4,3,3,3,
3,3,3,3,3,3,3,3,4),(0.,1.12535551671007E-5,7.76936938506112E-5,0.000102513517961138,
0.000121879189824284,0.000189659041345297,0.000223548967105804,0.000257294099096102,
0.000257438892866311,0.000325720851751308,0.000396486773947479,0.000466242707652249,
0.000514877785732621),.UNSPECIFIED.);
#4866=B_SPLINE_CURVE_WITH_KNOTS('',3,(#216618,#216619,#216620,#216621,#216622,
#216623,#216624,#216625,#216626,#216627,#216628,#216629,#216630,#216631,
#216632,#216633,#216634,#216635,#216636,#216637,#216638,#216639,#216640,
#216641,#216642,#216643,#216644,#216645,#216646,#216647,#216648,#216649,
#216650,#216651,#216652,#216653,#216654,#216655,#216656,#216657),
 .UNSPECIFIED.,.F.,.F.,(4,3,3,3,3,3,3,3,3,3,3,3,3,4),(0.,6.80370855331494E-5,
0.000137303169291901,0.000203636706654186,0.000256396220959702,0.000256540237295728,
0.000285209320207747,0.000342105100635661,0.000384776935956597,0.000400778874201948,
0.000456785658060676,0.00048478904999004,0.000498790745954722,0.000512792441919404),
 .UNSPECIFIED.);
#4867=B_SPLINE_CURVE_WITH_KNOTS('',3,(#216661,#216662,#216663,#216664,#216665,
#216666,#216667,#216668,#216669,#216670,#216671,#216672,#216673,#216674,
#216675,#216676,#216677,#216678,#216679,#216680,#216681,#216682,#216683,
#216684,#216685,#216686,#216687,#216688,#216689,#216690,#216691,#216692,
#216693,#216694,#216695,#216696,#216697),.UNSPECIFIED.,.F.,.F.,(4,3,3,3,
3,3,3,3,3,3,3,3,4),(0.,1.12535551670965E-5,7.76936938411505E-5,0.000102513517961098,
0.00012187918982425,0.00018965904134528,0.000223548967105795,0.000257294099096113,
0.00025743889286631,0.000325720851756961,0.00039648677395731,0.00046624270766338,
0.00051487778573262),.UNSPECIFIED.);
#4868=B_SPLINE_CURVE_WITH_KNOTS('',3,(#216705,#216706,#216707,#216708,#216709,
#216710,#216711,#216712,#216713,#216714,#216715,#216716,#216717,#216718,
#216719,#216720,#216721,#216722,#216723,#216724,#216725,#216726,#216727,
#216728,#216729,#216730,#216731,#216732,#216733,#216734,#216735,#216736,
#216737,#216738,#216739,#216740,#216741,#216742,#216743,#216744),
 .UNSPECIFIED.,.F.,.F.,(4,3,3,3,3,3,3,3,3,3,3,3,3,4),(0.,6.8037085541185E-5,
0.000137303169307903,0.000203636706677904,0.000256396220959706,0.000256540237295741,
0.00028520932020772,0.000342105100635643,0.000384776935956585,0.000400778874201939,
0.000456785658060676,0.000484789049990044,0.000498790745954728,0.000512792441919413),
 .UNSPECIFIED.);
#4869=B_SPLINE_CURVE_WITH_KNOTS('',3,(#216748,#216749,#216750,#216751,#216752,
#216753,#216754,#216755,#216756,#216757,#216758,#216759,#216760,#216761,
#216762,#216763,#216764,#216765,#216766,#216767,#216768,#216769,#216770,
#216771,#216772,#216773,#216774,#216775,#216776,#216777,#216778,#216779,
#216780,#216781,#216782,#216783,#216784),.UNSPECIFIED.,.F.,.F.,(4,3,3,3,
3,3,3,3,3,3,3,3,4),(0.,1.12535551670995E-5,7.76936938413587E-5,0.000102513517961138,
0.000121879189824285,0.0001896590413453,0.000223548967105808,0.00025729409909611,
0.000257438892866315,0.000325720851766884,0.000396486773977355,0.000466242707691934,
0.00051487778573263),.UNSPECIFIED.);
#4870=B_SPLINE_CURVE_WITH_KNOTS('',3,(#216792,#216793,#216794,#216795,#216796,
#216797,#216798,#216799,#216800,#216801,#216802,#216803,#216804,#216805,
#216806,#216807,#216808,#216809,#216810,#216811,#216812,#216813,#216814,
#216815,#216816,#216817,#216818,#216819,#216820,#216821,#216822,#216823,
#216824,#216825,#216826,#216827,#216828,#216829,#216830,#216831),
 .UNSPECIFIED.,.F.,.F.,(4,3,3,3,3,3,3,3,3,3,3,3,3,4),(0.,6.80370855392613E-5,
0.000137303169304968,0.000203636706675208,0.000256396220959704,0.000256540237295727,
0.000285209320207745,0.000342105100635661,0.000384776935956598,0.000400778874201949,
0.000456785658060679,0.000484789049990044,0.000498790745954726,0.000512792441919408),
 .UNSPECIFIED.);
#4871=B_SPLINE_CURVE_WITH_KNOTS('',3,(#216835,#216836,#216837,#216838,#216839,
#216840,#216841,#216842,#216843,#216844,#216845,#216846,#216847,#216848,
#216849,#216850,#216851,#216852,#216853,#216854,#216855,#216856,#216857,
#216858,#216859,#216860,#216861,#216862,#216863,#216864,#216865,#216866,
#216867,#216868,#216869,#216870,#216871),.UNSPECIFIED.,.F.,.F.,(4,3,3,3,
3,3,3,3,3,3,3,3,4),(0.,1.1253555167103E-5,7.76936938409016E-5,0.000102513517961149,
0.000121879189824294,0.000189659041345302,0.000223548967105806,0.000257294099096109,
0.00025743889286631,0.00032572085175361,0.000396486773951826,0.000466242707658243,
0.000514877785732621),.UNSPECIFIED.);
#4872=B_SPLINE_CURVE_WITH_KNOTS('',3,(#216879,#216880,#216881,#216882,#216883,
#216884,#216885,#216886,#216887,#216888,#216889,#216890,#216891,#216892,
#216893,#216894,#216895,#216896,#216897,#216898,#216899,#216900,#216901,
#216902,#216903,#216904,#216905,#216906,#216907,#216908,#216909,#216910,
#216911,#216912,#216913,#216914,#216915,#216916,#216917,#216918),
 .UNSPECIFIED.,.F.,.F.,(4,3,3,3,3,3,3,3,3,3,3,3,3,4),(0.,6.80370855404509E-5,
0.000137303169306047,0.000203636706674211,0.000256396220959703,0.000256540237295742,
0.000285209320207733,0.000342105100635652,0.00038477693595659,0.000400778874201942,
0.000456785658060675,0.000484789049990041,0.000498790745954724,0.000512792441919407),
 .UNSPECIFIED.);
#4873=B_SPLINE_CURVE_WITH_KNOTS('',3,(#216922,#216923,#216924,#216925,#216926,
#216927,#216928,#216929,#216930,#216931,#216932,#216933,#216934,#216935,
#216936,#216937,#216938,#216939,#216940,#216941,#216942,#216943,#216944,
#216945,#216946,#216947,#216948,#216949,#216950,#216951,#216952,#216953,
#216954,#216955,#216956,#216957,#216958),.UNSPECIFIED.,.F.,.F.,(4,3,3,3,
3,3,3,3,3,3,3,3,4),(0.,1.12535551670926E-5,7.76936938578812E-5,0.000102513517961074,
0.000121879189824228,0.00018965904134527,0.00022354896710579,0.000257294099096107,
0.000257438892866311,0.000325720851755129,0.000396486773954983,0.000466242707662315,
0.000514877785732621),.UNSPECIFIED.);
#4874=B_SPLINE_CURVE_WITH_KNOTS('',3,(#216966,#216967,#216968,#216969,#216970,
#216971,#216972,#216973,#216974,#216975,#216976,#216977,#216978,#216979,
#216980,#216981,#216982,#216983,#216984,#216985,#216986,#216987,#216988,
#216989,#216990,#216991,#216992,#216993,#216994,#216995,#216996,#216997,
#216998,#216999,#217000,#217001,#217002,#217003,#217004,#217005),
 .UNSPECIFIED.,.F.,.F.,(4,3,3,3,3,3,3,3,3,3,3,3,3,4),(0.,6.80370855390923E-5,
0.000137303169303434,0.000203636706670414,0.000256396220959702,0.000256540237295738,
0.000285209320207726,0.000342105100635646,0.000384776935956586,0.000400778874201938,
0.000456785658060671,0.000484789049990038,0.000498790745954721,0.000512792441919405),
 .UNSPECIFIED.);
#4875=B_SPLINE_CURVE_WITH_KNOTS('',3,(#217009,#217010,#217011,#217012,#217013,
#217014,#217015,#217016,#217017,#217018,#217019,#217020,#217021,#217022,
#217023,#217024,#217025,#217026,#217027,#217028,#217029,#217030,#217031,
#217032,#217033,#217034,#217035,#217036,#217037,#217038,#217039,#217040,
#217041,#217042,#217043,#217044,#217045),.UNSPECIFIED.,.F.,.F.,(4,3,3,3,
3,3,3,3,3,3,3,3,4),(0.,1.12535551670967E-5,7.76936938457851E-5,0.000102513517961083,
0.000121879189824237,0.000189659041345273,0.000223548967105791,0.000257294099096112,
0.000257438892866309,0.000325720851758272,0.000396486773960363,0.000466242707668341,
0.000514877785732617),.UNSPECIFIED.);
#4876=B_SPLINE_CURVE_WITH_KNOTS('',3,(#217053,#217054,#217055,#217056,#217057,
#217058,#217059,#217060,#217061,#217062,#217063,#217064,#217065,#217066,
#217067,#217068,#217069,#217070,#217071,#217072,#217073,#217074,#217075,
#217076,#217077,#217078,#217079,#217080,#217081,#217082,#217083,#217084,
#217085,#217086,#217087,#217088,#217089,#217090,#217091,#217092),
 .UNSPECIFIED.,.F.,.F.,(4,3,3,3,3,3,3,3,3,3,3,3,3,4),(0.,6.80370855408783E-5,
0.000137303169307437,0.000203636706676985,0.000256396220959703,0.000256540237295734,
0.000285209320207724,0.000342105100635644,0.000384776935956585,0.000400778874201937,
0.000456785658060672,0.000484789049990039,0.000498790745954723,0.000512792441919406),
 .UNSPECIFIED.);
#4877=B_SPLINE_CURVE_WITH_KNOTS('',3,(#217096,#217097,#217098,#217099,#217100,
#217101,#217102,#217103,#217104,#217105,#217106,#217107,#217108,#217109,
#217110,#217111,#217112,#217113,#217114,#217115,#217116,#217117,#217118,
#217119,#217120,#217121,#217122,#217123,#217124,#217125,#217126,#217127,
#217128,#217129,#217130,#217131,#217132),.UNSPECIFIED.,.F.,.F.,(4,3,3,3,
3,3,3,3,3,3,3,3,4),(0.,1.12535551670943E-5,7.76936938418916E-5,0.000102513517961078,
0.000121879189824232,0.000189659041345268,0.000223548967105787,0.000257294099096112,
0.000257438892866305,0.000325720851760699,0.000396486773966138,0.000466242707678695,
0.00051487778573261),.UNSPECIFIED.);
#4878=B_SPLINE_CURVE_WITH_KNOTS('',3,(#217140,#217141,#217142,#217143,#217144,
#217145,#217146,#217147,#217148,#217149,#217150,#217151,#217152,#217153,
#217154,#217155,#217156,#217157,#217158,#217159,#217160,#217161,#217162,
#217163,#217164,#217165,#217166,#217167,#217168,#217169,#217170,#217171,
#217172,#217173,#217174,#217175,#217176,#217177,#217178,#217179),
 .UNSPECIFIED.,.F.,.F.,(4,3,3,3,3,3,3,3,3,3,3,3,3,4),(0.,6.80370855409884E-5,
0.000137303169307076,0.000203636706675499,0.000256396220959705,0.00025654023729574,
0.000285209320207724,0.000342105100635646,0.000384776935956587,0.00040077887420194,
0.000456785658060675,0.000484789049990042,0.000498790745954726,0.00051279244191941),
 .UNSPECIFIED.);
#4879=B_SPLINE_CURVE_WITH_KNOTS('',3,(#217183,#217184,#217185,#217186,#217187,
#217188,#217189,#217190,#217191,#217192,#217193,#217194,#217195,#217196,
#217197,#217198,#217199,#217200,#217201,#217202,#217203,#217204,#217205,
#217206,#217207,#217208,#217209,#217210,#217211,#217212,#217213,#217214,
#217215,#217216,#217217,#217218,#217219),.UNSPECIFIED.,.F.,.F.,(4,3,3,3,
3,3,3,3,3,3,3,3,4),(0.,1.12535551670965E-5,7.76936938395602E-5,0.000102513517961085,
0.000121879189824238,0.000189659041345273,0.000223548967105791,0.000257294099096104,
0.000257438892866308,0.000325720851759098,0.000396486773962644,0.000466242707673163,
0.000514877785732617),.UNSPECIFIED.);
#4880=B_SPLINE_CURVE_WITH_KNOTS('',3,(#217227,#217228,#217229,#217230,#217231,
#217232,#217233,#217234,#217235,#217236,#217237,#217238,#217239,#217240,
#217241,#217242,#217243,#217244,#217245,#217246,#217247,#217248,#217249,
#217250,#217251,#217252,#217253,#217254,#217255,#217256,#217257,#217258,
#217259,#217260,#217261,#217262,#217263,#217264,#217265,#217266),
 .UNSPECIFIED.,.F.,.F.,(4,3,3,3,3,3,3,3,3,3,3,3,3,4),(0.,6.80370855374658E-5,
0.000137303169300085,0.000203636706665282,0.000256396220959703,0.00025654023729573,
0.000285209320207737,0.000342105100635654,0.000384776935956592,0.000400778874201944,
0.000456785658060675,0.00048478904999004,0.000498790745954723,0.000512792441919406),
 .UNSPECIFIED.);
#4881=B_SPLINE_CURVE_WITH_KNOTS('',3,(#217270,#217271,#217272,#217273,#217274,
#217275,#217276,#217277,#217278,#217279,#217280,#217281,#217282,#217283,
#217284,#217285,#217286,#217287,#217288,#217289,#217290,#217291,#217292,
#217293,#217294,#217295,#217296,#217297,#217298,#217299,#217300,#217301,
#217302,#217303,#217304,#217305,#217306),.UNSPECIFIED.,.F.,.F.,(4,3,3,3,
3,3,3,3,3,3,3,3,4),(0.,1.12535551670993E-5,7.76936938487074E-5,0.000102513517961113,
0.000121879189824263,0.000189659041345285,0.000223548967105796,0.000257294099096103,
0.000257438892866307,0.000325720851757075,0.000396486773958827,0.000466242707667839,
0.000514877785732613),.UNSPECIFIED.);
#4882=B_SPLINE_CURVE_WITH_KNOTS('',3,(#217314,#217315,#217316,#217317,#217318,
#217319,#217320,#217321,#217322,#217323,#217324,#217325,#217326,#217327,
#217328,#217329,#217330,#217331,#217332,#217333,#217334,#217335,#217336,
#217337,#217338,#217339,#217340,#217341,#217342,#217343,#217344,#217345,
#217346,#217347,#217348,#217349,#217350,#217351,#217352,#217353),
 .UNSPECIFIED.,.F.,.F.,(4,3,3,3,3,3,3,3,3,3,3,3,3,4),(0.,6.80370855423606E-5,
0.00013730316931023,0.000203636706680789,0.000256396220959703,0.000256540237295728,
0.000285209320207732,0.00034210510063565,0.000384776935956589,0.000400778874201941,
0.000456785658060673,0.000484789049990039,0.000498790745954722,0.000512792441919405),
 .UNSPECIFIED.);
#4883=B_SPLINE_CURVE_WITH_KNOTS('',3,(#217357,#217358,#217359,#217360,#217361,
#217362,#217363,#217364,#217365,#217366,#217367,#217368,#217369,#217370,
#217371,#217372,#217373,#217374,#217375,#217376,#217377,#217378,#217379,
#217380,#217381,#217382,#217383,#217384,#217385,#217386,#217387,#217388,
#217389,#217390,#217391,#217392,#217393),.UNSPECIFIED.,.F.,.F.,(4,3,3,3,
3,3,3,3,3,3,3,3,4),(0.,1.1253555167105E-5,7.76936938446724E-5,0.000102513517961175,
0.000121879189824317,0.000189659041345312,0.00022354896710581,0.000257294099096104,
0.000257438892866308,0.000325720851757317,0.000396486773958935,0.000466242707667538,
0.000514877785732616),.UNSPECIFIED.);
#4884=B_SPLINE_CURVE_WITH_KNOTS('',3,(#217401,#217402,#217403,#217404,#217405,
#217406,#217407,#217408,#217409,#217410,#217411,#217412,#217413,#217414,
#217415,#217416,#217417,#217418,#217419,#217420,#217421,#217422,#217423,
#217424,#217425,#217426,#217427,#217428,#217429,#217430,#217431,#217432,
#217433,#217434,#217435,#217436,#217437,#217438,#217439,#217440),
 .UNSPECIFIED.,.F.,.F.,(4,3,3,3,3,3,3,3,3,3,3,3,3,4),(0.,6.80370855342187E-5,
0.000137303169293596,0.00020363670665595,0.000256396220959707,0.000256540237295735,
0.000285209320207739,0.000342105100635658,0.000384776935956597,0.000400778874201949,
0.000456785658060681,0.000484789049990047,0.000498790745954731,0.000512792441919414),
 .UNSPECIFIED.);
#4885=B_SPLINE_CURVE_WITH_KNOTS('',3,(#217444,#217445,#217446,#217447,#217448,
#217449,#217450,#217451,#217452,#217453,#217454,#217455,#217456,#217457,
#217458,#217459,#217460,#217461,#217462,#217463,#217464,#217465,#217466,
#217467,#217468,#217469,#217470,#217471,#217472,#217473,#217474,#217475,
#217476,#217477,#217478,#217479,#217480),.UNSPECIFIED.,.F.,.F.,(4,3,3,3,
3,3,3,3,3,3,3,3,4),(0.,1.12535551671E-5,7.76936938449809E-5,0.000102513517961145,
0.000121879189824289,0.000189659041345296,0.0002235489671058,0.000257294099096096,
0.000257438892866303,0.000325720851758823,0.000396486773962096,0.000466242707672159,
0.000514877785732606),.UNSPECIFIED.);
#4886=B_SPLINE_CURVE_WITH_KNOTS('',3,(#217488,#217489,#217490,#217491,#217492,
#217493,#217494,#217495,#217496,#217497,#217498,#217499,#217500,#217501,
#217502,#217503,#217504,#217505,#217506,#217507,#217508,#217509,#217510,
#217511,#217512,#217513,#217514,#217515,#217516,#217517,#217518,#217519,
#217520,#217521,#217522,#217523,#217524,#217525,#217526,#217527),
 .UNSPECIFIED.,.F.,.F.,(4,3,3,3,3,3,3,3,3,3,3,3,3,4),(0.,6.80370855354539E-5,
0.000137303169295957,0.000203636706659032,0.000256396220959704,0.000256540237295736,
0.000285209320207732,0.000342105100635651,0.00038477693595659,0.000400778874201942,
0.000456785658060675,0.000484789049990042,0.000498790745954725,0.000512792441919408),
 .UNSPECIFIED.);
#4887=B_SPLINE_CURVE_WITH_KNOTS('',3,(#217531,#217532,#217533,#217534,#217535,
#217536,#217537,#217538,#217539,#217540,#217541,#217542,#217543,#217544,
#217545,#217546,#217547,#217548,#217549,#217550,#217551,#217552,#217553,
#217554,#217555,#217556,#217557,#217558,#217559,#217560,#217561,#217562,
#217563,#217564,#217565,#217566,#217567),.UNSPECIFIED.,.F.,.F.,(4,3,3,3,
3,3,3,3,3,3,3,3,4),(0.,1.1253555167102E-5,7.76936938454641E-5,0.00010251351796113,
0.000121879189824277,0.00018965904134529,0.000223548967105796,0.000257294099096106,
0.000257438892866303,0.000325720851760651,0.000396486773965936,0.000466242707677974,
0.000514877785732606),.UNSPECIFIED.);
#4888=B_SPLINE_CURVE_WITH_KNOTS('',3,(#217575,#217576,#217577,#217578,#217579,
#217580,#217581,#217582,#217583,#217584,#217585,#217586,#217587,#217588,
#217589,#217590,#217591,#217592,#217593,#217594,#217595,#217596,#217597,
#217598,#217599,#217600,#217601,#217602,#217603,#217604,#217605,#217606,
#217607,#217608,#217609,#217610,#217611,#217612,#217613,#217614),
 .UNSPECIFIED.,.F.,.F.,(4,3,3,3,3,3,3,3,3,3,3,3,3,4),(0.,6.803708553663E-5,
0.000137303169298813,0.000203636706664354,0.000256396220959703,0.00025654023729573,
0.000285209320207739,0.000342105100635656,0.000384776935956593,0.000400778874201945,
0.000456785658060676,0.000484789049990041,0.000498790745954724,0.000512792441919407),
 .UNSPECIFIED.);
#4889=B_SPLINE_CURVE_WITH_KNOTS('',3,(#217618,#217619,#217620,#217621,#217622,
#217623,#217624,#217625,#217626,#217627,#217628,#217629,#217630,#217631,
#217632,#217633,#217634,#217635,#217636,#217637,#217638,#217639,#217640,
#217641,#217642,#217643,#217644,#217645,#217646,#217647,#217648,#217649,
#217650,#217651,#217652,#217653,#217654),.UNSPECIFIED.,.F.,.F.,(4,3,3,3,
3,3,3,3,3,3,3,3,4),(0.,1.12535551671007E-5,7.76936938461026E-5,0.000102513517961134,
0.000121879189824281,0.000189659041345296,0.000223548967105803,0.000257294099096114,
0.00025743889286631,0.000325720851760575,0.000396486773965635,0.00046624270767721,
0.00051487778573262),.UNSPECIFIED.);
#4890=B_SPLINE_CURVE_WITH_KNOTS('',3,(#217662,#217663,#217664,#217665,#217666,
#217667,#217668,#217669,#217670,#217671,#217672,#217673,#217674,#217675,
#217676,#217677,#217678,#217679,#217680,#217681,#217682,#217683,#217684,
#217685,#217686,#217687,#217688,#217689,#217690,#217691,#217692,#217693,
#217694,#217695,#217696,#217697,#217698,#217699,#217700,#217701),
 .UNSPECIFIED.,.F.,.F.,(4,3,3,3,3,3,3,3,3,3,3,3,3,4),(0.,6.80370855347069E-5,
0.000137303169294128,0.000203636706655648,0.000256396220959708,0.000256540237295743,
0.000285209320207736,0.000342105100635656,0.000384776935956596,0.000400778874201949,
0.000456785658060683,0.000484789049990049,0.000498790745954733,0.000512792441919416),
 .UNSPECIFIED.);
#4891=B_SPLINE_CURVE_WITH_KNOTS('',3,(#217705,#217706,#217707,#217708,#217709,
#217710,#217711,#217712,#217713,#217714,#217715,#217716,#217717,#217718,
#217719,#217720,#217721,#217722,#217723,#217724,#217725,#217726,#217727,
#217728,#217729,#217730,#217731,#217732,#217733,#217734,#217735,#217736,
#217737,#217738,#217739,#217740,#217741),.UNSPECIFIED.,.F.,.F.,(4,3,3,3,
3,3,3,3,3,3,3,3,4),(0.,1.12535551670983E-5,7.76936938492197E-5,0.000102513517961119,
0.000121879189824267,0.000189659041345288,0.000223548967105798,0.000257294099096109,
0.000257438892866308,0.000325720851756761,0.000396486773957922,0.000466242707665982,
0.000514877785732616),.UNSPECIFIED.);
#4892=B_SPLINE_CURVE_WITH_KNOTS('',3,(#217749,#217750,#217751,#217752,#217753,
#217754,#217755,#217756,#217757,#217758,#217759,#217760,#217761,#217762,
#217763,#217764,#217765,#217766,#217767,#217768,#217769,#217770,#217771,
#217772,#217773,#217774,#217775,#217776,#217777,#217778,#217779,#217780,
#217781,#217782,#217783,#217784,#217785,#217786,#217787,#217788),
 .UNSPECIFIED.,.F.,.F.,(4,3,3,3,3,3,3,3,3,3,3,3,3,4),(0.,6.80370855408555E-5,
0.000137303169306811,0.000203636706674952,0.000256396220959707,0.000256540237295744,
0.000285209320207731,0.000342105100635651,0.000384776935956592,0.000400778874201945,
0.000456785658060679,0.000484789049990046,0.00049879074595473,0.000512792441919414),
 .UNSPECIFIED.);
#4893=B_SPLINE_CURVE_WITH_KNOTS('',3,(#217792,#217793,#217794,#217795,#217796,
#217797,#217798,#217799,#217800,#217801,#217802,#217803,#217804,#217805,
#217806,#217807,#217808,#217809,#217810,#217811,#217812,#217813,#217814,
#217815,#217816,#217817,#217818,#217819,#217820,#217821,#217822,#217823,
#217824,#217825,#217826,#217827,#217828),.UNSPECIFIED.,.F.,.F.,(4,3,3,3,
3,3,3,3,3,3,3,3,4),(0.,1.12535551670949E-5,7.76936938407407E-5,0.000102513517961092,
0.000121879189824244,0.000189659041345276,0.000223548967105792,0.00025729409909611,
0.000257438892866308,0.000325720851755195,0.000396486773954161,0.000466242707659613,
0.000514877785732615),.UNSPECIFIED.);
#4894=B_SPLINE_CURVE_WITH_KNOTS('',3,(#217836,#217837,#217838,#217839,#217840,
#217841,#217842,#217843,#217844,#217845,#217846,#217847,#217848,#217849,
#217850,#217851,#217852,#217853,#217854,#217855,#217856,#217857,#217858,
#217859,#217860,#217861,#217862,#217863,#217864,#217865,#217866,#217867,
#217868,#217869,#217870,#217871,#217872,#217873,#217874,#217875),
 .UNSPECIFIED.,.F.,.F.,(4,3,3,3,3,3,3,3,3,3,3,3,3,4),(0.,6.80370855333573E-5,
0.000137303169291925,0.000203636706653624,0.000256396220959706,0.000256540237295727,
0.000285209320207726,0.000342105100635648,0.000384776935956589,0.000400778874201942,
0.000456785658060677,0.000484789049990045,0.000498790745954729,0.000512792441919413),
 .UNSPECIFIED.);
#4895=B_SPLINE_CURVE_WITH_KNOTS('',3,(#217879,#217880,#217881,#217882,#217883,
#217884,#217885,#217886,#217887,#217888,#217889,#217890,#217891,#217892,
#217893,#217894,#217895,#217896,#217897,#217898,#217899,#217900,#217901,
#217902,#217903,#217904,#217905,#217906,#217907,#217908,#217909,#217910,
#217911,#217912,#217913,#217914,#217915),.UNSPECIFIED.,.F.,.F.,(4,3,3,3,
3,3,3,3,3,3,3,3,4),(0.,1.1253555167097E-5,7.76936938509154E-5,0.000102513517961086,
0.000121879189824237,0.000189659041345268,0.000223548967105783,0.000257294099096094,
0.000257438892866298,0.000325720851754246,0.000396486773952907,0.000466242707658961,
0.000514877785732597),.UNSPECIFIED.);
#4896=B_SPLINE_CURVE_WITH_KNOTS('',3,(#217923,#217924,#217925,#217926,#217927,
#217928,#217929,#217930,#217931,#217932,#217933,#217934,#217935,#217936,
#217937,#217938,#217939,#217940,#217941,#217942,#217943,#217944,#217945,
#217946,#217947,#217948,#217949,#217950,#217951,#217952,#217953,#217954,
#217955,#217956,#217957,#217958,#217959,#217960,#217961,#217962),
 .UNSPECIFIED.,.F.,.F.,(4,3,3,3,3,3,3,3,3,3,3,3,3,4),(0.,6.80370855338805E-5,
0.000137303169293391,0.000203636706656483,0.000256396220959711,0.000256540237295738,
0.000285209320207759,0.000342105100635674,0.000384776935956611,0.000400778874201962,
0.000456785658060692,0.000484789049990056,0.000498790745954739,0.000512792441919421),
 .UNSPECIFIED.);
#4897=B_SPLINE_CURVE_WITH_KNOTS('',3,(#217966,#217967,#217968,#217969,#217970,
#217971,#217972,#217973,#217974,#217975,#217976,#217977,#217978,#217979,
#217980,#217981,#217982,#217983,#217984,#217985,#217986,#217987,#217988,
#217989,#217990,#217991,#217992,#217993,#217994,#217995,#217996,#217997,
#217998,#217999,#218000,#218001,#218002),.UNSPECIFIED.,.F.,.F.,(4,3,3,3,
3,3,3,3,3,3,3,3,4),(0.,1.12535551670982E-5,7.769369384278E-5,0.000102513517961137,
0.000121879189824283,0.00018965904134529,0.000223548967105794,0.000257294099096092,
0.000257438892866298,0.000325720851758372,0.000396486773960825,0.000466242707669822,
0.000514877785732597),.UNSPECIFIED.);
#4898=B_SPLINE_CURVE_WITH_KNOTS('',3,(#218010,#218011,#218012,#218013,#218014,
#218015,#218016,#218017,#218018,#218019,#218020,#218021,#218022,#218023,
#218024,#218025,#218026,#218027,#218028,#218029,#218030,#218031,#218032,
#218033,#218034,#218035,#218036,#218037,#218038,#218039,#218040,#218041,
#218042,#218043,#218044,#218045,#218046,#218047,#218048,#218049),
 .UNSPECIFIED.,.F.,.F.,(4,3,3,3,3,3,3,3,3,3,3,3,3,4),(0.,6.80370855393617E-5,
0.000137303169304187,0.000203636706671761,0.000256396220959703,0.000256540237295725,
0.000285209320207727,0.000342105100635646,0.000384776935956586,0.000400778874201938,
0.000456785658060672,0.000484789049990039,0.000498790745954722,0.000512792441919405),
 .UNSPECIFIED.);
#4899=B_SPLINE_CURVE_WITH_KNOTS('',3,(#218053,#218054,#218055,#218056,#218057,
#218058,#218059,#218060,#218061,#218062,#218063,#218064,#218065,#218066,
#218067,#218068,#218069,#218070,#218071,#218072,#218073,#218074,#218075,
#218076,#218077,#218078,#218079,#218080,#218081,#218082,#218083,#218084,
#218085,#218086,#218087,#218088,#218089),.UNSPECIFIED.,.F.,.F.,(4,3,3,3,
3,3,3,3,3,3,3,3,4),(0.,1.12535551670974E-5,7.76936938354461E-5,0.000102513517961112,
0.000121879189824261,0.000189659041345284,0.000223548967105795,0.000257294099096103,
0.000257438892866306,0.000325720851764097,0.000396486773972469,0.000466242707686801,
0.000514877785732612),.UNSPECIFIED.);
#4900=B_SPLINE_CURVE_WITH_KNOTS('',3,(#218097,#218098,#218099,#218100,#218101,
#218102,#218103,#218104,#218105,#218106,#218107,#218108,#218109,#218110,
#218111,#218112,#218113,#218114,#218115,#218116,#218117,#218118,#218119,
#218120,#218121,#218122,#218123,#218124,#218125,#218126,#218127,#218128,
#218129,#218130,#218131,#218132,#218133,#218134,#218135,#218136),
 .UNSPECIFIED.,.F.,.F.,(4,3,3,3,3,3,3,3,3,3,3,3,3,4),(0.,6.8037085540861E-5,
0.000137303169307164,0.000203636706676043,0.000256396220959705,0.000256540237295742,
0.000285209320207739,0.000342105100635657,0.000384776935956595,0.000400778874201947,
0.000456785658060679,0.000484789049990045,0.000498790745954728,0.000512792441919411),
 .UNSPECIFIED.);
#4901=B_SPLINE_CURVE_WITH_KNOTS('',3,(#218140,#218141,#218142,#218143,#218144,
#218145,#218146,#218147,#218148,#218149,#218150,#218151,#218152,#218153,
#218154,#218155,#218156,#218157,#218158,#218159,#218160,#218161,#218162,
#218163,#218164,#218165,#218166,#218167,#218168,#218169,#218170,#218171,
#218172,#218173,#218174,#218175,#218176),.UNSPECIFIED.,.F.,.F.,(4,3,3,3,
3,3,3,3,3,3,3,3,4),(0.,1.12535551670985E-5,7.76936938454086E-5,0.000102513517961139,
0.000121879189824285,0.000189659041345297,0.000223548967105803,0.000257294099096096,
0.000257438892866308,0.000325720851768916,0.000396486773983027,0.000466242707703339,
0.000514877785732617),.UNSPECIFIED.);
#4902=B_SPLINE_CURVE_WITH_KNOTS('',3,(#218184,#218185,#218186,#218187,#218188,
#218189,#218190,#218191,#218192,#218193,#218194,#218195,#218196,#218197,
#218198,#218199,#218200,#218201,#218202,#218203,#218204,#218205,#218206,
#218207,#218208,#218209,#218210,#218211,#218212,#218213,#218214,#218215,
#218216,#218217,#218218,#218219,#218220,#218221,#218222,#218223),
 .UNSPECIFIED.,.F.,.F.,(4,3,3,3,3,3,3,3,3,3,3,3,3,4),(0.,6.80370855365877E-5,
0.000137303169299356,0.000203636706666889,0.000256396220959707,0.000256540237295743,
0.000285209320207725,0.000342105100635648,0.000384776935956589,0.000400778874201942,
0.000456785658060678,0.000484789049990046,0.00049879074595473,0.000512792441919414),
 .UNSPECIFIED.);
#4903=B_SPLINE_CURVE_WITH_KNOTS('',3,(#218227,#218228,#218229,#218230,#218231,
#218232,#218233,#218234,#218235,#218236,#218237,#218238,#218239,#218240,
#218241,#218242,#218243,#218244,#218245,#218246,#218247,#218248,#218249,
#218250,#218251,#218252,#218253,#218254,#218255,#218256,#218257,#218258,
#218259,#218260,#218261,#218262,#218263),.UNSPECIFIED.,.F.,.F.,(4,3,3,3,
3,3,3,3,3,3,3,3,4),(0.,1.12535551670997E-5,7.76936938459687E-5,0.000102513517961119,
0.000121879189824267,0.000189659041345284,0.000223548967105793,0.000257294099096094,
0.000257438892866301,0.000325720851764935,0.000396486773975291,0.000466242707692906,
0.000514877785732603),.UNSPECIFIED.);
#4904=B_SPLINE_CURVE_WITH_KNOTS('',3,(#218271,#218272,#218273,#218274,#218275,
#218276,#218277,#218278,#218279,#218280,#218281,#218282,#218283,#218284,
#218285,#218286,#218287,#218288,#218289,#218290,#218291,#218292,#218293,
#218294,#218295,#218296,#218297,#218298,#218299,#218300,#218301,#218302,
#218303,#218304,#218305,#218306,#218307,#218308,#218309,#218310),
 .UNSPECIFIED.,.F.,.F.,(4,3,3,3,3,3,3,3,3,3,3,3,3,4),(0.,6.80370855413805E-5,
0.000137303169307998,0.00020363670667671,0.000256396220959706,0.000256540237295745,
0.000285209320207745,0.000342105100635662,0.0003847769359566,0.000400778874201951,
0.000456785658060682,0.000484789049990047,0.00049879074595473,0.000512792441919413),
 .UNSPECIFIED.);
#4905=B_SPLINE_CURVE_WITH_KNOTS('',3,(#218314,#218315,#218316,#218317,#218318,
#218319,#218320,#218321,#218322,#218323,#218324,#218325,#218326,#218327,
#218328,#218329,#218330,#218331,#218332,#218333,#218334,#218335,#218336,
#218337,#218338,#218339,#218340,#218341,#218342,#218343,#218344,#218345,
#218346,#218347,#218348,#218349,#218350),.UNSPECIFIED.,.F.,.F.,(4,3,3,3,
3,3,3,3,3,3,3,3,4),(0.,1.12535551671018E-5,7.76936938515147E-5,0.000102513517961147,
0.000121879189824292,0.0001896590413453,0.000223548967105803,0.000257294099096102,
0.000257438892866307,0.000325720851754139,0.000396486773952012,0.000466242707656176,
0.000514877785732614),.UNSPECIFIED.);
#4906=B_SPLINE_CURVE_WITH_KNOTS('',3,(#218358,#218359,#218360,#218361,#218362,
#218363,#218364,#218365,#218366,#218367,#218368,#218369,#218370,#218371,
#218372,#218373,#218374,#218375,#218376,#218377,#218378,#218379,#218380,
#218381,#218382,#218383,#218384,#218385,#218386,#218387,#218388,#218389,
#218390,#218391,#218392,#218393,#218394,#218395,#218396,#218397),
 .UNSPECIFIED.,.F.,.F.,(4,3,3,3,3,3,3,3,3,3,3,3,3,4),(0.,6.80370855389298E-5,
0.000137303169302839,0.000203636706669121,0.000256396220959704,0.000256540237295741,
0.000285209320207746,0.000342105100635661,0.000384776935956598,0.000400778874201949,
0.000456785658060678,0.000484789049990043,0.000498790745954725,0.000512792441919407),
 .UNSPECIFIED.);
#4907=B_SPLINE_CURVE_WITH_KNOTS('',3,(#218401,#218402,#218403,#218404,#218405,
#218406,#218407,#218408,#218409,#218410,#218411,#218412,#218413,#218414,
#218415,#218416,#218417,#218418,#218419,#218420,#218421,#218422,#218423,
#218424,#218425,#218426,#218427,#218428,#218429,#218430,#218431,#218432,
#218433,#218434,#218435,#218436,#218437),.UNSPECIFIED.,.F.,.F.,(4,3,3,3,
3,3,3,3,3,3,3,3,4),(0.,1.12535551670959E-5,7.76936938459669E-5,0.0001025135179611,
0.00012187918982425,0.000189659041345275,0.000223548967105788,0.000257294099096094,
0.000257438892866301,0.000325720851752298,0.000396486773948228,0.000466242707650774,
0.000514877785732601),.UNSPECIFIED.);
#4908=B_SPLINE_CURVE_WITH_KNOTS('',3,(#218445,#218446,#218447,#218448,#218449,
#218450,#218451,#218452,#218453,#218454,#218455,#218456,#218457,#218458,
#218459,#218460,#218461,#218462,#218463,#218464,#218465,#218466,#218467,
#218468,#218469,#218470,#218471,#218472,#218473,#218474,#218475,#218476,
#218477,#218478,#218479,#218480,#218481,#218482,#218483,#218484),
 .UNSPECIFIED.,.F.,.F.,(4,3,3,3,3,3,3,3,3,3,3,3,3,4),(0.,6.80370855424441E-5,
0.000137303169309744,0.000203636706678789,0.000256396220959707,0.000256540237295729,
0.000285209320207743,0.000342105100635661,0.000384776935956599,0.000400778874201951,
0.000456785658060683,0.000484789049990049,0.000498790745954732,0.000512792441919415),
 .UNSPECIFIED.);
#4909=B_SPLINE_CURVE_WITH_KNOTS('',3,(#218488,#218489,#218490,#218491,#218492,
#218493,#218494,#218495,#218496,#218497,#218498,#218499,#218500,#218501,
#218502,#218503,#218504,#218505,#218506,#218507,#218508,#218509,#218510,
#218511,#218512,#218513,#218514,#218515,#218516,#218517,#218518,#218519,
#218520,#218521,#218522,#218523,#218524),.UNSPECIFIED.,.F.,.F.,(4,3,3,3,
3,3,3,3,3,3,3,3,4),(0.,1.12535551670972E-5,7.76936938431592E-5,0.00010251351796109,
0.000121879189824242,0.000189659041345273,0.000223548967105789,0.000257294099096099,
0.000257438892866304,0.000325720851758791,0.000396486773961801,0.000466242707671268,
0.000514877785732608),.UNSPECIFIED.);
#4910=B_SPLINE_CURVE_WITH_KNOTS('',3,(#218532,#218533,#218534,#218535,#218536,
#218537,#218538,#218539,#218540,#218541,#218542,#218543,#218544,#218545,
#218546,#218547,#218548,#218549,#218550,#218551,#218552,#218553,#218554,
#218555,#218556,#218557,#218558,#218559,#218560,#218561,#218562,#218563,
#218564,#218565,#218566,#218567,#218568,#218569,#218570,#218571),
 .UNSPECIFIED.,.F.,.F.,(4,3,3,3,3,3,3,3,3,3,3,3,3,4),(0.,6.8037085534851E-5,
0.000137303169294966,0.000203636706658237,0.000256396220959703,0.000256540237295729,
0.000285209320207737,0.000342105100635654,0.000384776935956592,0.000400778874201944,
0.000456785658060675,0.00048478904999004,0.000498790745954723,0.000512792441919405),
 .UNSPECIFIED.);
#4911=B_SPLINE_CURVE_WITH_KNOTS('',3,(#218575,#218576,#218577,#218578,#218579,
#218580,#218581,#218582,#218583,#218584,#218585,#218586,#218587,#218588,
#218589,#218590,#218591,#218592,#218593,#218594,#218595,#218596,#218597,
#218598,#218599,#218600,#218601,#218602,#218603,#218604,#218605,#218606,
#218607,#218608,#218609,#218610,#218611),.UNSPECIFIED.,.F.,.F.,(4,3,3,3,
3,3,3,3,3,3,3,3,4),(0.,1.12535551670989E-5,7.76936938479744E-5,0.000102513517961094,
0.000121879189824246,0.000189659041345275,0.00022354896710579,0.000257294099096105,
0.000257438892866304,0.00032572085175291,0.000396486773950194,0.000466242707655154,
0.000514877785732609),.UNSPECIFIED.);
#4912=B_SPLINE_CURVE_WITH_KNOTS('',3,(#218619,#218620,#218621,#218622,#218623,
#218624,#218625,#218626,#218627,#218628,#218629,#218630,#218631,#218632,
#218633,#218634,#218635,#218636,#218637,#218638,#218639,#218640,#218641,
#218642,#218643,#218644,#218645,#218646,#218647,#218648,#218649,#218650,
#218651,#218652,#218653,#218654,#218655,#218656,#218657,#218658),
 .UNSPECIFIED.,.F.,.F.,(4,3,3,3,3,3,3,3,3,3,3,3,3,4),(0.,6.80370855361618E-5,
0.000137303169297681,0.000203636706662249,0.000256396220959705,0.000256540237295736,
0.000285209320207737,0.000342105100635655,0.000384776935956594,0.000400778874201946,
0.000456785658060677,0.000484789049990043,0.000498790745954726,0.000512792441919409),
 .UNSPECIFIED.);
#4913=B_SPLINE_CURVE_WITH_KNOTS('',3,(#218662,#218663,#218664,#218665,#218666,
#218667,#218668,#218669,#218670,#218671,#218672,#218673,#218674,#218675,
#218676,#218677,#218678,#218679,#218680,#218681,#218682,#218683,#218684,
#218685,#218686,#218687,#218688,#218689,#218690,#218691,#218692,#218693,
#218694,#218695,#218696,#218697,#218698),.UNSPECIFIED.,.F.,.F.,(4,3,3,3,
3,3,3,3,3,3,3,3,4),(0.,1.12535551671016E-5,7.76936938480596E-5,0.000102513517961156,
0.0001218791898243,0.000189659041345303,0.000223548967105804,0.000257294099096105,
0.000257438892866306,0.000325720851759106,0.000396486773962859,0.00046624270767365,
0.000514877785732612),.UNSPECIFIED.);
#4914=B_SPLINE_CURVE_WITH_KNOTS('',3,(#218706,#218707,#218708,#218709,#218710,
#218711,#218712,#218713,#218714,#218715,#218716,#218717,#218718,#218719,
#218720,#218721,#218722,#218723,#218724,#218725,#218726,#218727,#218728,
#218729,#218730,#218731,#218732,#218733,#218734,#218735,#218736,#218737,
#218738,#218739,#218740,#218741,#218742,#218743,#218744,#218745),
 .UNSPECIFIED.,.F.,.F.,(4,3,3,3,3,3,3,3,3,3,3,3,3,4),(0.,6.8037085534625E-5,
0.00013730316929443,0.000203636706657177,0.000256396220959704,0.000256540237295729,
0.000285209320207743,0.00034210510063566,0.000384776935956597,0.000400778874201948,
0.000456785658060678,0.000484789049990043,0.000498790745954726,0.000512792441919408),
 .UNSPECIFIED.);
#4915=B_SPLINE_CURVE_WITH_KNOTS('',3,(#218752,#218753,#218754,#218755,#218756,
#218757,#218758,#218759,#218760,#218761,#218762,#218763,#218764,#218765,
#218766,#218767,#218768,#218769,#218770,#218771,#218772,#218773,#218774,
#218775,#218776,#218777,#218778,#218779,#218780,#218781,#218782,#218783,
#218784,#218785,#218786,#218787,#218788),.UNSPECIFIED.,.F.,.F.,(4,3,3,3,
3,3,3,3,3,3,3,3,4),(0.,1.12535551670991E-5,7.76936938497371E-5,0.000102513517961127,
0.000121879189824275,0.00018965904134529,0.000223548967105798,0.000257294099096094,
0.000257438892866306,0.000325720851756744,0.000396486773957958,0.000466242707666199,
0.000514877785732612),.UNSPECIFIED.);
#4916=B_SPLINE_CURVE_WITH_KNOTS('',3,(#218796,#218797,#218798,#218799,#218800,
#218801,#218802,#218803,#218804,#218805,#218806,#218807,#218808,#218809,
#218810,#218811,#218812,#218813,#218814,#218815,#218816,#218817,#218818,
#218819,#218820,#218821,#218822,#218823,#218824,#218825,#218826,#218827,
#218828,#218829,#218830,#218831,#218832,#218833,#218834,#218835),
 .UNSPECIFIED.,.F.,.F.,(4,3,3,3,3,3,3,3,3,3,3,3,3,4),(0.,6.8037085536429E-5,
0.00013730316929818,0.000203636706662896,0.000256396220959701,0.000256540237295736,
0.000285209320207738,0.000342105100635654,0.000384776935956591,0.000400778874201942,
0.000456785658060672,0.000484789049990037,0.000498790745954719,0.000512792441919401),
 .UNSPECIFIED.);
#4917=B_SPLINE_CURVE_WITH_KNOTS('',3,(#218839,#218840,#218841,#218842,#218843,
#218844,#218845,#218846,#218847,#218848,#218849,#218850,#218851,#218852,
#218853,#218854,#218855,#218856,#218857,#218858,#218859,#218860,#218861,
#218862,#218863,#218864,#218865,#218866,#218867,#218868,#218869,#218870,
#218871,#218872,#218873,#218874,#218875),.UNSPECIFIED.,.F.,.F.,(4,3,3,3,
3,3,3,3,3,3,3,3,4),(0.,1.12535551670982E-5,7.76936938451034E-5,0.000102513517961114,
0.000121879189824263,0.000189659041345285,0.000223548967105796,0.000257294099096108,
0.000257438892866307,0.000325720851759771,0.000396486773963886,0.000466242707674355,
0.000514877785732613),.UNSPECIFIED.);
#4918=B_SPLINE_CURVE_WITH_KNOTS('',3,(#218883,#218884,#218885,#218886,#218887,
#218888,#218889,#218890,#218891,#218892,#218893,#218894,#218895,#218896,
#218897,#218898,#218899,#218900,#218901,#218902,#218903,#218904,#218905,
#218906,#218907,#218908,#218909,#218910,#218911,#218912,#218913,#218914,
#218915,#218916,#218917,#218918,#218919,#218920,#218921,#218922),
 .UNSPECIFIED.,.F.,.F.,(4,3,3,3,3,3,3,3,3,3,3,3,3,4),(0.,6.80370855360243E-5,
0.000137303169297593,0.000203636706662558,0.000256396220959703,0.000256540237295725,
0.000285209320207735,0.000342105100635653,0.000384776935956591,0.000400778874201943,
0.000456785658060674,0.00048478904999004,0.000498790745954723,0.000512792441919406),
 .UNSPECIFIED.);
#4919=B_SPLINE_CURVE_WITH_KNOTS('',3,(#218926,#218927,#218928,#218929,#218930,
#218931,#218932,#218933,#218934,#218935,#218936,#218937,#218938,#218939,
#218940,#218941,#218942,#218943,#218944,#218945,#218946,#218947,#218948,
#218949,#218950,#218951,#218952,#218953,#218954,#218955,#218956,#218957,
#218958,#218959,#218960,#218961,#218962),.UNSPECIFIED.,.F.,.F.,(4,3,3,3,
3,3,3,3,3,3,3,3,4),(0.,1.12535551670984E-5,7.76936938487798E-5,0.000102513517961109,
0.000121879189824259,0.000189659041345282,0.000223548967105794,0.000257294099096103,
0.000257438892866306,0.000325720851760856,0.000396486773966341,0.000466242707678374,
0.000514877785732612),.UNSPECIFIED.);
#4920=B_SPLINE_CURVE_WITH_KNOTS('',3,(#218970,#218971,#218972,#218973,#218974,
#218975,#218976,#218977,#218978,#218979,#218980,#218981,#218982,#218983,
#218984,#218985,#218986,#218987,#218988,#218989,#218990,#218991,#218992,
#218993,#218994,#218995,#218996,#218997,#218998,#218999,#219000,#219001,
#219002,#219003,#219004,#219005,#219006,#219007,#219008,#219009),
 .UNSPECIFIED.,.F.,.F.,(4,3,3,3,3,3,3,3,3,3,3,3,3,4),(0.,6.80370855341084E-5,
0.000137303169293612,0.000203636706656273,0.000256396220959707,0.000256540237295736,
0.000285209320207752,0.000342105100635667,0.000384776935956604,0.000400778874201955,
0.000456785658060684,0.000484789049990049,0.000498790745954731,0.000512792441919413),
 .UNSPECIFIED.);
#4921=B_SPLINE_CURVE_WITH_KNOTS('',3,(#219013,#219014,#219015,#219016,#219017,
#219018,#219019,#219020,#219021,#219022,#219023,#219024,#219025,#219026,
#219027,#219028,#219029,#219030,#219031,#219032,#219033,#219034,#219035,
#219036,#219037,#219038,#219039,#219040,#219041,#219042,#219043,#219044,
#219045,#219046,#219047,#219048,#219049),.UNSPECIFIED.,.F.,.F.,(4,3,3,3,
3,3,3,3,3,3,3,3,4),(0.,1.1253555167101E-5,7.76936938410561E-5,0.000102513517961155,
0.000121879189824298,0.000189659041345302,0.000223548967105803,0.000257294099096109,
0.000257438892866305,0.000325720851758758,0.000396486773962038,0.000466242707672476,
0.000514877785732609),.UNSPECIFIED.);
#4922=B_SPLINE_CURVE_WITH_KNOTS('',3,(#219057,#219058,#219059,#219060,#219061,
#219062,#219063,#219064,#219065,#219066,#219067,#219068,#219069,#219070,
#219071,#219072,#219073,#219074,#219075,#219076,#219077,#219078,#219079,
#219080,#219081,#219082,#219083,#219084,#219085,#219086,#219087,#219088,
#219089,#219090,#219091,#219092,#219093,#219094,#219095,#219096),
 .UNSPECIFIED.,.F.,.F.,(4,3,3,3,3,3,3,3,3,3,3,3,3,4),(0.,6.80370855362772E-5,
0.0001373031692974,0.000203636706660765,0.000256396220959705,0.00025654023729573,
0.000285209320207733,0.000342105100635652,0.000384776935956592,0.000400778874201944,
0.000456785658060677,0.000484789049990043,0.000498790745954727,0.00051279244191941),
 .UNSPECIFIED.);
#4923=B_SPLINE_CURVE_WITH_KNOTS('',3,(#219100,#219101,#219102,#219103,#219104,
#219105,#219106,#219107,#219108,#219109,#219110,#219111,#219112,#219113,
#219114,#219115,#219116,#219117,#219118,#219119,#219120,#219121,#219122,
#219123,#219124,#219125,#219126,#219127,#219128,#219129,#219130,#219131,
#219132,#219133,#219134,#219135,#219136),.UNSPECIFIED.,.F.,.F.,(4,3,3,3,
3,3,3,3,3,3,3,3,4),(0.,1.12535551670954E-5,7.7693693843438E-5,0.000102513517961085,
0.000121879189824238,0.000189659041345273,0.000223548967105791,0.000257294099096106,
0.000257438892866309,0.0003257208517587,0.000396486773961633,0.000466242707671069,
0.000514877785732617),.UNSPECIFIED.);
#4924=B_SPLINE_CURVE_WITH_KNOTS('',3,(#219144,#219145,#219146,#219147,#219148,
#219149,#219150,#219151,#219152,#219153,#219154,#219155,#219156,#219157,
#219158,#219159,#219160,#219161,#219162,#219163,#219164,#219165,#219166,
#219167,#219168,#219169,#219170,#219171,#219172,#219173,#219174,#219175,
#219176,#219177,#219178,#219179,#219180,#219181,#219182,#219183),
 .UNSPECIFIED.,.F.,.F.,(4,3,3,3,3,3,3,3,3,3,3,3,3,4),(0.,6.80370855369493E-5,
0.00013730316929952,0.000203636706665799,0.000256396220959709,0.000256540237295725,
0.000285209320207727,0.00034210510063565,0.000384776935956592,0.000400778874201945,
0.000456785658060681,0.000484789049990049,0.000498790745954733,0.000512792441919417),
 .UNSPECIFIED.);
#4925=B_SPLINE_CURVE_WITH_KNOTS('',3,(#219187,#219188,#219189,#219190,#219191,
#219192,#219193,#219194,#219195,#219196,#219197,#219198,#219199,#219200,
#219201,#219202,#219203,#219204,#219205,#219206,#219207,#219208,#219209,
#219210,#219211,#219212,#219213,#219214,#219215,#219216,#219217,#219218,
#219219,#219220,#219221,#219222,#219223),.UNSPECIFIED.,.F.,.F.,(4,3,3,3,
3,3,3,3,3,3,3,3,4),(0.,1.12535551670973E-5,7.76936938503403E-5,0.000102513517961109,
0.000121879189824258,0.000189659041345281,0.000223548967105792,0.000257294099096104,
0.000257438892866303,0.000325720851751885,0.000396486773948232,0.000466242707652404,
0.000514877785732606),.UNSPECIFIED.);
#4926=B_SPLINE_CURVE_WITH_KNOTS('',3,(#219231,#219232,#219233,#219234,#219235,
#219236,#219237,#219238,#219239,#219240,#219241,#219242,#219243,#219244,
#219245,#219246,#219247,#219248,#219249,#219250,#219251,#219252,#219253,
#219254,#219255,#219256,#219257,#219258,#219259,#219260,#219261,#219262,
#219263,#219264,#219265,#219266,#219267,#219268,#219269,#219270),
 .UNSPECIFIED.,.F.,.F.,(4,3,3,3,3,3,3,3,3,3,3,3,3,4),(0.,6.80370855305542E-5,
0.000137303169286892,0.000203636706647725,0.000256396220959703,0.000256540237295726,
0.00028520932020773,0.000342105100635649,0.000384776935956589,0.000400778874201941,
0.000456785658060674,0.00048478904999004,0.000498790745954723,0.000512792441919407),
 .UNSPECIFIED.);
#4927=B_SPLINE_CURVE_WITH_KNOTS('',3,(#219274,#219275,#219276,#219277,#219278,
#219279,#219280,#219281,#219282,#219283,#219284,#219285,#219286,#219287,
#219288,#219289,#219290,#219291,#219292,#219293,#219294,#219295,#219296,
#219297,#219298,#219299,#219300,#219301,#219302,#219303,#219304,#219305,
#219306,#219307,#219308,#219309,#219310),.UNSPECIFIED.,.F.,.F.,(4,3,3,3,
3,3,3,3,3,3,3,3,4),(0.,1.12535551670967E-5,7.7693693841938E-5,0.000102513517961121,
0.000121879189824269,0.000189659041345287,0.000223548967105796,0.000257294099096099,
0.000257438892866305,0.000325720851753896,0.000396486773952486,0.000466242707659185,
0.000514877785732609),.UNSPECIFIED.);
#4928=B_SPLINE_CURVE_WITH_KNOTS('',3,(#219318,#219319,#219320,#219321,#219322,
#219323,#219324,#219325,#219326,#219327,#219328,#219329,#219330,#219331,
#219332,#219333,#219334,#219335,#219336,#219337,#219338,#219339,#219340,
#219341,#219342,#219343,#219344,#219345,#219346,#219347,#219348,#219349,
#219350,#219351,#219352,#219353,#219354,#219355,#219356,#219357),
 .UNSPECIFIED.,.F.,.F.,(4,3,3,3,3,3,3,3,3,3,3,3,3,4),(0.,6.80370855360398E-5,
0.000137303169296802,0.000203636706659669,0.000256396220959709,0.000256540237295733,
0.00028520932020774,0.000342105100635659,0.000384776935956599,0.000400778874201952,
0.000456785658060685,0.000484789049990052,0.000498790745954735,0.000512792441919418),
 .UNSPECIFIED.);
#4929=B_SPLINE_CURVE_WITH_KNOTS('',3,(#219361,#219362,#219363,#219364,#219365,
#219366,#219367,#219368,#219369,#219370,#219371,#219372,#219373,#219374,
#219375,#219376,#219377,#219378,#219379,#219380,#219381,#219382,#219383,
#219384,#219385,#219386,#219387,#219388,#219389,#219390,#219391,#219392,
#219393,#219394,#219395,#219396,#219397),.UNSPECIFIED.,.F.,.F.,(4,3,3,3,
3,3,3,3,3,3,3,3,4),(0.,1.12535551671021E-5,7.76936938520304E-5,0.00010251351796116,
0.000121879189824304,0.000189659041345306,0.000223548967105807,0.00025729409909611,
0.000257438892866308,0.00032572085175869,0.000396486773962042,0.000466242707672318,
0.000514877785732615),.UNSPECIFIED.);
#4930=B_SPLINE_CURVE_WITH_KNOTS('',3,(#219405,#219406,#219407,#219408,#219409,
#219410,#219411,#219412,#219413,#219414,#219415,#219416,#219417,#219418,
#219419,#219420,#219421,#219422,#219423,#219424,#219425,#219426,#219427,
#219428,#219429,#219430,#219431,#219432,#219433,#219434,#219435,#219436,
#219437,#219438,#219439,#219440,#219441,#219442,#219443,#219444),
 .UNSPECIFIED.,.F.,.F.,(4,3,3,3,3,3,3,3,3,3,3,3,3,4),(0.,6.80370855343923E-5,
0.000137303169294156,0.000203636706657648,0.000256396220959702,0.00025654023729573,
0.000285209320207731,0.000342105100635649,0.000384776935956587,0.000400778874201939,
0.000456785658060671,0.000484789049990037,0.00049879074595472,0.000512792441919403),
 .UNSPECIFIED.);
#4931=B_SPLINE_CURVE_WITH_KNOTS('',3,(#219448,#219449,#219450,#219451,#219452,
#219453,#219454,#219455,#219456,#219457,#219458,#219459,#219460,#219461,
#219462,#219463,#219464,#219465,#219466,#219467,#219468,#219469,#219470,
#219471,#219472,#219473,#219474,#219475,#219476,#219477,#219478,#219479,
#219480,#219481,#219482,#219483,#219484),.UNSPECIFIED.,.F.,.F.,(4,3,3,3,
3,3,3,3,3,3,3,3,4),(0.,1.12535551671044E-5,7.76936938363717E-5,0.000102513517961159,
0.000121879189824302,0.000189659041345305,0.000223548967105807,0.000257294099096106,
0.000257438892866309,0.00032572085175684,0.000396486773958732,0.000466242707668953,
0.000514877785732617),.UNSPECIFIED.);
#4932=B_SPLINE_CURVE_WITH_KNOTS('',3,(#219492,#219493,#219494,#219495,#219496,
#219497,#219498,#219499,#219500,#219501,#219502,#219503,#219504,#219505,
#219506,#219507,#219508,#219509,#219510,#219511,#219512,#219513,#219514,
#219515,#219516,#219517,#219518,#219519,#219520,#219521,#219522,#219523,
#219524,#219525,#219526,#219527,#219528,#219529,#219530,#219531),
 .UNSPECIFIED.,.F.,.F.,(4,3,3,3,3,3,3,3,3,3,3,3,3,4),(0.,6.80370855361023E-5,
0.000137303169297632,0.00020363670666265,0.000256396220959704,0.000256540237295734,
0.000285209320207739,0.000342105100635657,0.000384776935956595,0.000400778874201946,
0.000456785658060677,0.000484789049990043,0.000498790745954726,0.000512792441919408),
 .UNSPECIFIED.);
#4933=B_SPLINE_CURVE_WITH_KNOTS('',3,(#219535,#219536,#219537,#219538,#219539,
#219540,#219541,#219542,#219543,#219544,#219545,#219546,#219547,#219548,
#219549,#219550,#219551,#219552,#219553,#219554,#219555,#219556,#219557,
#219558,#219559,#219560,#219561,#219562,#219563,#219564,#219565,#219566,
#219567,#219568,#219569,#219570,#219571),.UNSPECIFIED.,.F.,.F.,(4,3,3,3,
3,3,3,3,3,3,3,3,4),(0.,1.12535551671001E-5,7.76936938493738E-5,0.000102513517961137,
0.000121879189824282,0.000189659041345291,0.000223548967105795,0.000257294099096098,
0.000257438892866299,0.00032572085174627,0.000396486773936295,0.000466242707634075,
0.000514877785732599),.UNSPECIFIED.);
#4934=B_SPLINE_CURVE_WITH_KNOTS('',3,(#219579,#219580,#219581,#219582,#219583,
#219584,#219585,#219586,#219587,#219588,#219589,#219590,#219591,#219592,
#219593,#219594,#219595,#219596,#219597,#219598,#219599,#219600,#219601,
#219602,#219603,#219604,#219605,#219606,#219607,#219608,#219609,#219610,
#219611,#219612,#219613,#219614,#219615,#219616,#219617,#219618),
 .UNSPECIFIED.,.F.,.F.,(4,3,3,3,3,3,3,3,3,3,3,3,3,4),(0.,6.80370855373009E-5,
0.000137303169299663,0.000203636706664318,0.000256396220959702,0.000256540237295726,
0.000285209320207732,0.00034210510063565,0.000384776935956588,0.00040077887420194,
0.000456785658060672,0.000484789049990038,0.000498790745954721,0.000512792441919404),
 .UNSPECIFIED.);
#4935=B_SPLINE_CURVE_WITH_KNOTS('',3,(#219622,#219623,#219624,#219625,#219626,
#219627,#219628,#219629,#219630,#219631,#219632,#219633,#219634,#219635,
#219636,#219637,#219638,#219639,#219640,#219641,#219642,#219643,#219644,
#219645,#219646,#219647,#219648,#219649,#219650,#219651,#219652,#219653,
#219654,#219655,#219656,#219657,#219658),.UNSPECIFIED.,.F.,.F.,(4,3,3,3,
3,3,3,3,3,3,3,3,4),(0.,1.12535551670992E-5,7.76936938444347E-5,0.000102513517961116,
0.000121879189824265,0.000189659041345288,0.000223548967105799,0.000257294099096112,
0.00025743889286631,0.00032572085175845,0.000396486773961124,0.000466242707670346,
0.000514877785732621),.UNSPECIFIED.);
#4936=B_SPLINE_CURVE_WITH_KNOTS('',3,(#219666,#219667,#219668,#219669,#219670,
#219671,#219672,#219673,#219674,#219675,#219676,#219677,#219678,#219679,
#219680,#219681,#219682,#219683,#219684,#219685,#219686,#219687,#219688,
#219689,#219690,#219691,#219692,#219693,#219694,#219695,#219696,#219697,
#219698,#219699,#219700,#219701,#219702,#219703,#219704,#219705),
 .UNSPECIFIED.,.F.,.F.,(4,3,3,3,3,3,3,3,3,3,3,3,3,4),(0.,6.80370855375739E-5,
0.000137303169299986,0.000203636706664461,0.000256396220959699,0.000256540237295735,
0.000285209320207733,0.00034210510063565,0.000384776935956587,0.000400778874201938,
0.000456785658060669,0.000484789049990034,0.000498790745954716,0.000512792441919399),
 .UNSPECIFIED.);
#4937=B_SPLINE_CURVE_WITH_KNOTS('',3,(#219709,#219710,#219711,#219712,#219713,
#219714,#219715,#219716,#219717,#219718,#219719,#219720,#219721,#219722,
#219723,#219724,#219725,#219726,#219727,#219728,#219729,#219730,#219731,
#219732,#219733,#219734,#219735,#219736,#219737,#219738,#219739,#219740,
#219741,#219742,#219743,#219744,#219745),.UNSPECIFIED.,.F.,.F.,(4,3,3,3,
3,3,3,3,3,3,3,3,4),(0.,1.12535551671018E-5,7.76936938560993E-5,0.000102513517961127,
0.000121879189824273,0.000189659041345284,0.00022354896710579,0.000257294099096101,
0.000257438892866296,0.00032572085175287,0.000396486773949805,0.000466242707653759,
0.000514877785732592),.UNSPECIFIED.);
#4938=B_SPLINE_CURVE_WITH_KNOTS('',3,(#219753,#219754,#219755,#219756,#219757,
#219758,#219759,#219760,#219761,#219762,#219763,#219764,#219765,#219766,
#219767,#219768,#219769,#219770,#219771,#219772,#219773,#219774,#219775,
#219776,#219777,#219778,#219779,#219780,#219781,#219782,#219783,#219784,
#219785,#219786,#219787,#219788,#219789,#219790,#219791,#219792),
 .UNSPECIFIED.,.F.,.F.,(4,3,3,3,3,3,3,3,3,3,3,3,3,4),(0.,6.80370855373682E-5,
0.00013730316930006,0.000203636706665804,0.000256396220959704,0.000256540237295727,
0.000285209320207723,0.000342105100635644,0.000384776935956585,0.000400778874201938,
0.000456785658060672,0.00048478904999004,0.000498790745954723,0.000512792441919407),
 .UNSPECIFIED.);
#4939=B_SPLINE_CURVE_WITH_KNOTS('',3,(#219796,#219797,#219798,#219799,#219800,
#219801,#219802,#219803,#219804,#219805,#219806,#219807,#219808,#219809,
#219810,#219811,#219812,#219813,#219814,#219815,#219816,#219817,#219818,
#219819,#219820,#219821,#219822,#219823,#219824,#219825,#219826,#219827,
#219828,#219829,#219830,#219831,#219832),.UNSPECIFIED.,.F.,.F.,(4,3,3,3,
3,3,3,3,3,3,3,3,4),(0.,1.12535551670959E-5,7.7693693848883E-5,0.000102513517961114,
0.000121879189824263,0.000189659041345284,0.000223548967105795,0.000257294099096117,
0.000257438892866305,0.000325720851755243,0.000396486773954683,0.000466242707661072,
0.00051487778573261),.UNSPECIFIED.);
#4940=B_SPLINE_CURVE_WITH_KNOTS('',3,(#219840,#219841,#219842,#219843,#219844,
#219845,#219846,#219847,#219848,#219849,#219850,#219851,#219852,#219853,
#219854,#219855,#219856,#219857,#219858,#219859,#219860,#219861,#219862,
#219863,#219864,#219865,#219866,#219867,#219868,#219869,#219870,#219871,
#219872,#219873,#219874,#219875,#219876,#219877,#219878,#219879),
 .UNSPECIFIED.,.F.,.F.,(4,3,3,3,3,3,3,3,3,3,3,3,3,4),(0.,6.80370855356864E-5,
0.000137303169296884,0.000203636706661411,0.000256396220959704,0.00025654023729573,
0.00028520932020772,0.000342105100635642,0.000384776935956584,0.000400778874201937,
0.000456785658060672,0.00048478904999004,0.000498790745954724,0.000512792441919408),
 .UNSPECIFIED.);
#4941=B_SPLINE_CURVE_WITH_KNOTS('',3,(#219883,#219884,#219885,#219886,#219887,
#219888,#219889,#219890,#219891,#219892,#219893,#219894,#219895,#219896,
#219897,#219898,#219899,#219900,#219901,#219902,#219903,#219904,#219905,
#219906,#219907,#219908,#219909,#219910,#219911,#219912,#219913,#219914,
#219915,#219916,#219917,#219918,#219919),.UNSPECIFIED.,.F.,.F.,(4,3,3,3,
3,3,3,3,3,3,3,3,4),(0.,1.12535551670985E-5,7.76936938457793E-5,0.000102513517961143,
0.000121879189824288,0.000189659041345298,0.000223548967105802,0.0002572940990961,
0.000257438892866307,0.000325720851758952,0.000396486773962268,0.00046624270767231,
0.000514877785732614),.UNSPECIFIED.);
#4942=B_SPLINE_CURVE_WITH_KNOTS('',3,(#219927,#219928,#219929,#219930,#219931,
#219932,#219933,#219934,#219935,#219936,#219937,#219938,#219939,#219940,
#219941,#219942,#219943,#219944,#219945,#219946,#219947,#219948,#219949,
#219950,#219951,#219952,#219953,#219954,#219955,#219956,#219957,#219958,
#219959,#219960,#219961,#219962,#219963,#219964,#219965,#219966),
 .UNSPECIFIED.,.F.,.F.,(4,3,3,3,3,3,3,3,3,3,3,3,3,4),(0.,6.80370855404787E-5,
0.000137303169306344,0.000203636706674795,0.000256396220959704,0.000256540237295735,
0.000285209320207736,0.000342105100635654,0.000384776935956593,0.000400778874201945,
0.000456785658060677,0.000484789049990043,0.000498790745954726,0.000512792441919409),
 .UNSPECIFIED.);
#4943=B_SPLINE_CURVE_WITH_KNOTS('',3,(#219970,#219971,#219972,#219973,#219974,
#219975,#219976,#219977,#219978,#219979,#219980,#219981,#219982,#219983,
#219984,#219985,#219986,#219987,#219988,#219989,#219990,#219991,#219992,
#219993,#219994,#219995,#219996,#219997,#219998,#219999,#220000,#220001,
#220002,#220003,#220004,#220005,#220006),.UNSPECIFIED.,.F.,.F.,(4,3,3,3,
3,3,3,3,3,3,3,3,4),(0.,1.12535551670986E-5,7.76936938445697E-5,0.000102513517961116,
0.000121879189824264,0.000189659041345283,0.000223548967105793,0.00025729409909611,
0.000257438892866302,0.000325720851758691,0.000396486773961759,0.000466242707671471,
0.000514877785732605),.UNSPECIFIED.);
#4944=B_SPLINE_CURVE_WITH_KNOTS('',3,(#220013,#220014,#220015,#220016,#220017,
#220018,#220019,#220020,#220021,#220022,#220023,#220024,#220025,#220026,
#220027,#220028,#220029,#220030,#220031,#220032,#220033,#220034,#220035,
#220036,#220037,#220038,#220039,#220040,#220041,#220042,#220043,#220044,
#220045,#220046,#220047,#220048,#220049,#220050,#220051,#220052),
 .UNSPECIFIED.,.F.,.F.,(4,3,3,3,3,3,3,3,3,3,3,3,3,4),(0.,6.80370855342381E-5,
0.000137303169293626,0.000203636706655953,0.000256396220959707,0.00025654023729573,
0.000285209320207736,0.000342105100635655,0.000384776935956595,0.000400778874201947,
0.00045678565806068,0.000484789049990047,0.00049879074595473,0.000512792441919414),
 .UNSPECIFIED.);
#4945=B_SPLINE_CURVE_WITH_KNOTS('',3,(#220054,#220055,#220056,#220057,#220058,
#220059,#220060,#220061,#220062,#220063,#220064,#220065,#220066,#220067,
#220068,#220069,#220070,#220071,#220072,#220073,#220074,#220075,#220076,
#220077,#220078,#220079,#220080,#220081,#220082,#220083,#220084,#220085,
#220086,#220087,#220088,#220089,#220090),.UNSPECIFIED.,.F.,.F.,(4,3,3,3,
3,3,3,3,3,3,3,3,4),(0.,1.12535551671018E-5,7.76936938435877E-5,0.000102513517961135,
0.000121879189824281,0.000189659041345292,0.000223548967105798,0.000257294099096097,
0.000257438892866303,0.000325720851759153,0.000396486773962767,0.000466242707673162,
0.000514877785732606),.UNSPECIFIED.);
#4946=B_SPLINE_CURVE_WITH_KNOTS('',3,(#220098,#220099,#220100,#220101,#220102,
#220103,#220104,#220105,#220106,#220107,#220108,#220109,#220110,#220111,
#220112,#220113,#220114,#220115,#220116,#220117,#220118,#220119,#220120,
#220121,#220122,#220123,#220124,#220125,#220126,#220127,#220128,#220129,
#220130,#220131,#220132,#220133,#220134,#220135,#220136,#220137),
 .UNSPECIFIED.,.F.,.F.,(4,3,3,3,3,3,3,3,3,3,3,3,3,4),(0.,6.80370855408103E-5,
0.000137303169307113,0.000203636706676278,0.000256396220959706,0.000256540237295737,
0.00028520932020774,0.000342105100635658,0.000384776935956596,0.000400778874201948,
0.00045678565806068,0.000484789049990046,0.000498790745954729,0.000512792441919412),
 .UNSPECIFIED.);
#4947=B_SPLINE_CURVE_WITH_KNOTS('',3,(#220141,#220142,#220143,#220144,#220145,
#220146,#220147,#220148,#220149,#220150,#220151,#220152,#220153,#220154,
#220155,#220156,#220157,#220158,#220159,#220160,#220161,#220162,#220163,
#220164,#220165,#220166,#220167,#220168,#220169,#220170,#220171,#220172,
#220173,#220174,#220175,#220176,#220177),.UNSPECIFIED.,.F.,.F.,(4,3,3,3,
3,3,3,3,3,3,3,3,4),(0.,1.12535551670972E-5,7.76936938468974E-5,0.000102513517961115,
0.000121879189824263,0.000189659041345284,0.000223548967105794,0.000257294099096101,
0.000257438892866304,0.000325720851754898,0.000396486773954035,0.000466242707660405,
0.000514877785732608),.UNSPECIFIED.);
#4948=B_SPLINE_CURVE_WITH_KNOTS('',3,(#220185,#220186,#220187,#220188,#220189,
#220190,#220191,#220192,#220193,#220194,#220195,#220196,#220197,#220198,
#220199,#220200,#220201,#220202,#220203,#220204,#220205,#220206,#220207,
#220208,#220209,#220210,#220211,#220212,#220213,#220214,#220215,#220216,
#220217,#220218,#220219,#220220,#220221,#220222,#220223,#220224),
 .UNSPECIFIED.,.F.,.F.,(4,3,3,3,3,3,3,3,3,3,3,3,3,4),(0.,6.80370855378567E-5,
0.000137303169300862,0.000203636706666544,0.000256396220959703,0.000256540237295736,
0.000285209320207733,0.000342105100635651,0.00038477693595659,0.000400778874201942,
0.000456785658060673,0.000484789049990039,0.000498790745954722,0.000512792441919405),
 .UNSPECIFIED.);
#4949=B_SPLINE_CURVE_WITH_KNOTS('',3,(#220228,#220229,#220230,#220231,#220232,
#220233,#220234,#220235,#220236,#220237,#220238,#220239,#220240,#220241,
#220242,#220243,#220244,#220245,#220246,#220247,#220248,#220249,#220250,
#220251,#220252,#220253,#220254,#220255,#220256,#220257,#220258,#220259,
#220260,#220261,#220262,#220263,#220264),.UNSPECIFIED.,.F.,.F.,(4,3,3,3,
3,3,3,3,3,3,3,3,4),(0.,1.12535551670993E-5,7.76936938400127E-5,0.00010251351796113,
0.000121879189824277,0.000189659041345292,0.000223548967105799,0.000257294099096103,
0.000257438892866306,0.000325720851756268,0.000396486773956665,0.000466242707663886,
0.000514877785732613),.UNSPECIFIED.);
#4950=B_SPLINE_CURVE_WITH_KNOTS('',3,(#220272,#220273,#220274,#220275,#220276,
#220277,#220278,#220279,#220280,#220281,#220282,#220283,#220284,#220285,
#220286,#220287,#220288,#220289,#220290,#220291,#220292,#220293,#220294,
#220295,#220296,#220297,#220298,#220299,#220300,#220301,#220302,#220303,
#220304,#220305,#220306,#220307,#220308,#220309,#220310,#220311),
 .UNSPECIFIED.,.F.,.F.,(4,3,3,3,3,3,3,3,3,3,3,3,3,4),(0.,6.80370855365677E-5,
0.000137303169297886,0.000203636706661229,0.000256396220959701,0.000256540237295728,
0.00028520932020773,0.000342105100635649,0.000384776935956587,0.000400778874201939,
0.000456785658060671,0.000484789049990037,0.00049879074595472,0.000512792441919403),
 .UNSPECIFIED.);
#4951=B_SPLINE_CURVE_WITH_KNOTS('',3,(#220315,#220316,#220317,#220318,#220319,
#220320,#220321,#220322,#220323,#220324,#220325,#220326,#220327,#220328,
#220329,#220330,#220331,#220332,#220333,#220334,#220335,#220336,#220337,
#220338,#220339,#220340,#220341,#220342,#220343,#220344,#220345,#220346,
#220347,#220348,#220349,#220350,#220351),.UNSPECIFIED.,.F.,.F.,(4,3,3,3,
3,3,3,3,3,3,3,3,4),(0.,1.12535551670979E-5,7.76936938450434E-5,0.000102513517961105,
0.000121879189824256,0.000189659041345283,0.000223548967105797,0.00025729409909611,
0.000257438892866311,0.000325720851755806,0.000396486773955716,0.000466242707662355,
0.000514877785732622),.UNSPECIFIED.);
#4952=B_SPLINE_CURVE_WITH_KNOTS('',3,(#220359,#220360,#220361,#220362,#220363,
#220364,#220365,#220366,#220367,#220368,#220369,#220370,#220371,#220372,
#220373,#220374,#220375,#220376,#220377,#220378,#220379,#220380,#220381,
#220382,#220383,#220384,#220385,#220386,#220387,#220388,#220389,#220390,
#220391,#220392,#220393,#220394,#220395,#220396,#220397,#220398),
 .UNSPECIFIED.,.F.,.F.,(4,3,3,3,3,3,3,3,3,3,3,3,3,4),(0.,6.80370855353079E-5,
0.000137303169296173,0.000203636706660593,0.0002563962209597,0.000256540237295731,
0.000285209320207733,0.000342105100635649,0.000384776935956587,0.000400778874201939,
0.000456785658060669,0.000484789049990034,0.000498790745954717,0.0005127924419194),
 .UNSPECIFIED.);
#4953=B_SPLINE_CURVE_WITH_KNOTS('',3,(#220402,#220403,#220404,#220405,#220406,
#220407,#220408,#220409,#220410,#220411,#220412,#220413,#220414,#220415,
#220416,#220417,#220418,#220419,#220420,#220421,#220422,#220423,#220424,
#220425,#220426,#220427,#220428,#220429,#220430,#220431,#220432,#220433,
#220434,#220435,#220436,#220437,#220438),.UNSPECIFIED.,.F.,.F.,(4,3,3,3,
3,3,3,3,3,3,3,3,4),(0.,1.12535551670958E-5,7.76936938484934E-5,0.0001025135179611,
0.000121879189824251,0.000189659041345279,0.000223548967105793,0.000257294099096104,
0.000257438892866307,0.00032572085176472,0.000396486773974065,0.000466242707689337,
0.000514877785732614),.UNSPECIFIED.);
#4954=B_SPLINE_CURVE_WITH_KNOTS('',3,(#220446,#220447,#220448,#220449,#220450,
#220451,#220452,#220453,#220454,#220455,#220456,#220457,#220458,#220459,
#220460,#220461,#220462,#220463,#220464,#220465,#220466,#220467,#220468,
#220469,#220470,#220471,#220472,#220473,#220474,#220475,#220476,#220477,
#220478,#220479,#220480,#220481,#220482,#220483,#220484,#220485),
 .UNSPECIFIED.,.F.,.F.,(4,3,3,3,3,3,3,3,3,3,3,3,3,4),(0.,6.80370855370149E-5,
0.000137303169299152,0.00020363670666395,0.000256396220959702,0.000256540237295726,
0.000285209320207733,0.000342105100635651,0.000384776935956589,0.000400778874201941,
0.000456785658060673,0.000484789049990039,0.000498790745954722,0.000512792441919404),
 .UNSPECIFIED.);
#4955=B_SPLINE_CURVE_WITH_KNOTS('',3,(#220489,#220490,#220491,#220492,#220493,
#220494,#220495,#220496,#220497,#220498,#220499,#220500,#220501,#220502,
#220503,#220504,#220505,#220506,#220507,#220508,#220509,#220510,#220511,
#220512,#220513,#220514,#220515,#220516,#220517,#220518,#220519,#220520,
#220521,#220522,#220523,#220524,#220525),.UNSPECIFIED.,.F.,.F.,(4,3,3,3,
3,3,3,3,3,3,3,3,4),(0.,1.12535551670976E-5,7.76936938539417E-5,0.000102513517961119,
0.000121879189824268,0.000189659041345289,0.0002235489671058,0.000257294099096114,
0.00025743889286631,0.000325720851758913,0.000396486773961676,0.000466242707670145,
0.000514877785732621),.UNSPECIFIED.);
#4956=B_SPLINE_CURVE_WITH_KNOTS('',3,(#220533,#220534,#220535,#220536,#220537,
#220538,#220539,#220540,#220541,#220542,#220543,#220544,#220545,#220546,
#220547,#220548,#220549,#220550,#220551,#220552,#220553,#220554,#220555,
#220556,#220557,#220558,#220559,#220560,#220561,#220562,#220563,#220564,
#220565,#220566,#220567,#220568,#220569,#220570,#220571,#220572),
 .UNSPECIFIED.,.F.,.F.,(4,3,3,3,3,3,3,3,3,3,3,3,3,4),(0.,6.80370855405262E-5,
0.000137303169306291,0.000203636706674482,0.000256396220959699,0.000256540237295709,
0.000285209320207743,0.000342105100635657,0.000384776935956592,0.000400778874201943,
0.00045678565806067,0.000484789049990034,0.000498790745954716,0.000512792441919397),
 .UNSPECIFIED.);
#4957=B_SPLINE_CURVE_WITH_KNOTS('',3,(#220576,#220577,#220578,#220579,#220580,
#220581,#220582,#220583,#220584,#220585,#220586,#220587,#220588,#220589,
#220590,#220591,#220592,#220593,#220594,#220595,#220596,#220597,#220598,
#220599,#220600,#220601,#220602,#220603,#220604,#220605,#220606,#220607,
#220608,#220609,#220610,#220611,#220612),.UNSPECIFIED.,.F.,.F.,(4,3,3,3,
3,3,3,3,3,3,3,3,4),(0.,1.12535551670982E-5,7.7693693851138E-5,0.000102513517961117,
0.000121879189824266,0.000189659041345289,0.0002235489671058,0.000257294099096116,
0.000257438892866312,0.000325720851754073,0.000396486773952516,0.000466242707658386,
0.000514877785732623),.UNSPECIFIED.);
#4958=B_SPLINE_CURVE_WITH_KNOTS('',3,(#220620,#220621,#220622,#220623,#220624,
#220625,#220626,#220627,#220628,#220629,#220630,#220631,#220632,#220633,
#220634,#220635,#220636,#220637,#220638,#220639,#220640,#220641,#220642,
#220643,#220644,#220645,#220646,#220647,#220648,#220649,#220650,#220651,
#220652,#220653,#220654,#220655,#220656,#220657,#220658,#220659),
 .UNSPECIFIED.,.F.,.F.,(4,3,3,3,3,3,3,3,3,3,3,3,3,4),(0.,6.80370855406125E-5,
0.000137303169307245,0.000203636706678069,0.000256396220959702,0.000256540237295741,
0.000285209320207742,0.000342105100635658,0.000384776935956594,0.000400778874201945,
0.000456785658060675,0.000484789049990039,0.000498790745954721,0.000512792441919404),
 .UNSPECIFIED.);
#4959=B_SPLINE_CURVE_WITH_KNOTS('',3,(#220663,#220664,#220665,#220666,#220667,
#220668,#220669,#220670,#220671,#220672,#220673,#220674,#220675,#220676,
#220677,#220678,#220679,#220680,#220681,#220682,#220683,#220684,#220685,
#220686,#220687,#220688,#220689,#220690,#220691,#220692,#220693,#220694,
#220695,#220696,#220697,#220698,#220699),.UNSPECIFIED.,.F.,.F.,(4,3,3,3,
3,3,3,3,3,3,3,3,4),(0.,1.12535551670976E-5,7.76936938533714E-5,0.000102513517961116,
0.000121879189824266,0.000189659041345289,0.000223548967105801,0.000257294099096104,
0.000257438892866313,0.000325720851754926,0.000396486773953946,0.000466242707659578,
0.000514877785732626),.UNSPECIFIED.);
#4960=B_SPLINE_CURVE_WITH_KNOTS('',3,(#220707,#220708,#220709,#220710,#220711,
#220712,#220713,#220714,#220715,#220716,#220717,#220718,#220719,#220720,
#220721,#220722,#220723,#220724,#220725,#220726,#220727,#220728,#220729,
#220730,#220731,#220732,#220733,#220734,#220735,#220736,#220737,#220738,
#220739,#220740,#220741,#220742,#220743,#220744,#220745,#220746),
 .UNSPECIFIED.,.F.,.F.,(4,3,3,3,3,3,3,3,3,3,3,3,3,4),(0.,6.80370855376524E-5,
0.000137303169300624,0.000203636706666611,0.000256396220959709,0.000256540237295741,
0.000285209320207731,0.000342105100635653,0.000384776935956595,0.000400778874201948,
0.000456785658060683,0.000484789049990051,0.000498790745954735,0.000512792441919419),
 .UNSPECIFIED.);
#4961=B_SPLINE_CURVE_WITH_KNOTS('',3,(#220750,#220751,#220752,#220753,#220754,
#220755,#220756,#220757,#220758,#220759,#220760,#220761,#220762,#220763,
#220764,#220765,#220766,#220767,#220768,#220769,#220770,#220771,#220772,
#220773,#220774,#220775,#220776,#220777,#220778,#220779,#220780,#220781,
#220782,#220783,#220784,#220785,#220786),.UNSPECIFIED.,.F.,.F.,(4,3,3,3,
3,3,3,3,3,3,3,3,4),(0.,1.12535551671015E-5,7.76936938364543E-5,0.000102513517961143,
0.000121879189824288,0.000189659041345293,0.000223548967105796,0.000257294099096091,
0.000257438892866299,0.000325720851761098,0.000396486773965608,0.000466242707675163,
0.000514877785732598),.UNSPECIFIED.);
#4962=B_SPLINE_CURVE_WITH_KNOTS('',3,(#220794,#220795,#220796,#220797,#220798,
#220799,#220800,#220801,#220802,#220803,#220804,#220805,#220806,#220807,
#220808,#220809,#220810,#220811,#220812,#220813,#220814,#220815,#220816,
#220817,#220818,#220819,#220820,#220821,#220822,#220823,#220824,#220825,
#220826,#220827,#220828,#220829,#220830,#220831,#220832,#220833),
 .UNSPECIFIED.,.F.,.F.,(4,3,3,3,3,3,3,3,3,3,3,3,3,4),(0.,6.80370855383874E-5,
0.000137303169301691,0.000203636706667116,0.000256396220959699,0.000256540237295735,
0.000285209320207737,0.000342105100635652,0.000384776935956589,0.00040077887420194,
0.000456785658060669,0.000484789049990033,0.000498790745954715,0.000512792441919398),
 .UNSPECIFIED.);
#4963=B_SPLINE_CURVE_WITH_KNOTS('',3,(#220837,#220838,#220839,#220840,#220841,
#220842,#220843,#220844,#220845,#220846,#220847,#220848,#220849,#220850,
#220851,#220852,#220853,#220854,#220855,#220856,#220857,#220858,#220859,
#220860,#220861,#220862,#220863,#220864,#220865,#220866,#220867,#220868,
#220869,#220870,#220871,#220872,#220873),.UNSPECIFIED.,.F.,.F.,(4,3,3,3,
3,3,3,3,3,3,3,3,4),(0.,1.1253555167099E-5,7.76936938505077E-5,0.000102513517961127,
0.000121879189824275,0.000189659041345293,0.000223548967105801,0.000257294099096114,
0.00025743889286631,0.000325720851755436,0.000396486773954861,0.00046624270766092,
0.000514877785732621),.UNSPECIFIED.);
#4964=B_SPLINE_CURVE_WITH_KNOTS('',3,(#220881,#220882,#220883,#220884,#220885,
#220886,#220887,#220888,#220889,#220890,#220891,#220892,#220893,#220894,
#220895,#220896,#220897,#220898,#220899,#220900,#220901,#220902,#220903,
#220904,#220905,#220906,#220907,#220908,#220909,#220910,#220911,#220912,
#220913,#220914,#220915,#220916,#220917,#220918,#220919,#220920),
 .UNSPECIFIED.,.F.,.F.,(4,3,3,3,3,3,3,3,3,3,3,3,3,4),(0.,6.80370855367628E-5,
0.000137303169298667,0.000203636706663435,0.000256396220959711,0.000256540237295747,
0.000285209320207732,0.000342105100635654,0.000384776935956596,0.000400778874201949,
0.000456785658060685,0.000484789049990053,0.000498790745954737,0.000512792441919421),
 .UNSPECIFIED.);
#4965=B_SPLINE_CURVE_WITH_KNOTS('',3,(#220924,#220925,#220926,#220927,#220928,
#220929,#220930,#220931,#220932,#220933,#220934,#220935,#220936,#220937,
#220938,#220939,#220940,#220941,#220942,#220943,#220944,#220945,#220946,
#220947,#220948,#220949,#220950,#220951,#220952,#220953,#220954,#220955,
#220956,#220957,#220958,#220959,#220960),.UNSPECIFIED.,.F.,.F.,(4,3,3,3,
3,3,3,3,3,3,3,3,4),(0.,1.12535551671004E-5,7.76936938370177E-5,0.000102513517961122,
0.00012187918982427,0.000189659041345288,0.000223548967105797,0.000257294099096105,
0.000257438892866306,0.000325720851761926,0.000396486773968017,0.000466242707679974,
0.000514877785732611),.UNSPECIFIED.);
#4966=B_SPLINE_CURVE_WITH_KNOTS('',3,(#220968,#220969,#220970,#220971,#220972,
#220973,#220974,#220975,#220976,#220977,#220978,#220979,#220980,#220981,
#220982,#220983,#220984,#220985,#220986,#220987,#220988,#220989,#220990,
#220991,#220992,#220993,#220994,#220995,#220996,#220997,#220998,#220999,
#221000,#221001,#221002,#221003,#221004,#221005,#221006,#221007),
 .UNSPECIFIED.,.F.,.F.,(4,3,3,3,3,3,3,3,3,3,3,3,3,4),(0.,6.80370855368759E-5,
0.000137303169298515,0.000203636706662323,0.000256396220959706,0.000256540237295727,
0.000285209320207712,0.000342105100635637,0.000384776935956581,0.000400778874201935,
0.000456785658060674,0.000484789049990043,0.000498790745954728,0.000512792441919413),
 .UNSPECIFIED.);
#4967=B_SPLINE_CURVE_WITH_KNOTS('',3,(#221011,#221012,#221013,#221014,#221015,
#221016,#221017,#221018,#221019,#221020,#221021,#221022,#221023,#221024,
#221025,#221026,#221027,#221028,#221029,#221030,#221031,#221032,#221033,
#221034,#221035,#221036,#221037,#221038,#221039,#221040,#221041,#221042,
#221043,#221044,#221045,#221046,#221047),.UNSPECIFIED.,.F.,.F.,(4,3,3,3,
3,3,3,3,3,3,3,3,4),(0.,1.12535551670969E-5,7.76936938444744E-5,0.000102513517961099,
0.000121879189824249,0.000189659041345277,0.00022354896710579,0.000257294099096095,
0.000257438892866304,0.000325720851753951,0.000396486773952143,0.000466242707657648,
0.000514877785732608),.UNSPECIFIED.);
#4968=B_SPLINE_CURVE_WITH_KNOTS('',3,(#221055,#221056,#221057,#221058,#221059,
#221060,#221061,#221062,#221063,#221064,#221065,#221066,#221067,#221068,
#221069,#221070,#221071,#221072,#221073,#221074,#221075,#221076,#221077,
#221078,#221079,#221080,#221081,#221082,#221083,#221084,#221085,#221086,
#221087,#221088,#221089,#221090,#221091,#221092,#221093,#221094),
 .UNSPECIFIED.,.F.,.F.,(4,3,3,3,3,3,3,3,3,3,3,3,3,4),(0.,6.80370855430361E-5,
0.000137303169311202,0.000203636706681394,0.000256396220959711,0.000256540237295744,
0.000285209320207742,0.000342105100635662,0.000384776935956602,0.000400778874201954,
0.000456785658060688,0.000484789049990054,0.000498790745954738,0.000512792441919421),
 .UNSPECIFIED.);
#4969=B_SPLINE_CURVE_WITH_KNOTS('',3,(#221098,#221099,#221100,#221101,#221102,
#221103,#221104,#221105,#221106,#221107,#221108,#221109,#221110,#221111,
#221112,#221113,#221114,#221115,#221116,#221117,#221118,#221119,#221120,
#221121,#221122,#221123,#221124,#221125,#221126,#221127,#221128,#221129,
#221130,#221131,#221132,#221133,#221134),.UNSPECIFIED.,.F.,.F.,(4,3,3,3,
3,3,3,3,3,3,3,3,4),(0.,1.12535551670993E-5,7.76936938391851E-5,0.000102513517961135,
0.000121879189824282,0.000189659041345295,0.000223548967105801,0.000257294099096109,
0.000257438892866308,0.000325720851757329,0.000396486773959131,0.000466242707668275,
0.000514877785732615),.UNSPECIFIED.);
#4970=B_SPLINE_CURVE_WITH_KNOTS('',3,(#221142,#221143,#221144,#221145,#221146,
#221147,#221148,#221149,#221150,#221151,#221152,#221153,#221154,#221155,
#221156,#221157,#221158,#221159,#221160,#221161,#221162,#221163,#221164,
#221165,#221166,#221167,#221168,#221169,#221170,#221171,#221172,#221173,
#221174,#221175,#221176,#221177,#221178,#221179,#221180,#221181),
 .UNSPECIFIED.,.F.,.F.,(4,3,3,3,3,3,3,3,3,3,3,3,3,4),(0.,6.80370855362148E-5,
0.000137303169297774,0.000203636706662515,0.000256396220959708,0.000256540237295738,
0.000285209320207736,0.000342105100635656,0.000384776935956596,0.000400778874201949,
0.000456785658060683,0.00048478904999005,0.000498790745954733,0.000512792441919417),
 .UNSPECIFIED.);
#4971=B_SPLINE_CURVE_WITH_KNOTS('',3,(#221185,#221186,#221187,#221188,#221189,
#221190,#221191,#221192,#221193,#221194,#221195,#221196,#221197,#221198,
#221199,#221200,#221201,#221202,#221203,#221204,#221205,#221206,#221207,
#221208,#221209,#221210,#221211,#221212,#221213,#221214,#221215,#221216,
#221217,#221218,#221219,#221220,#221221),.UNSPECIFIED.,.F.,.F.,(4,3,3,3,
3,3,3,3,3,3,3,3,4),(0.,1.12535551670964E-5,7.76936938562025E-5,0.0001025135179611,
0.00012187918982425,0.000189659041345276,0.000223548967105789,0.000257294099096091,
0.000257438892866302,0.00032572085175626,0.000396486773956917,0.000466242707664596,
0.000514877785732604),.UNSPECIFIED.);
#4972=B_SPLINE_CURVE_WITH_KNOTS('',3,(#221229,#221230,#221231,#221232,#221233,
#221234,#221235,#221236,#221237,#221238,#221239,#221240,#221241,#221242,
#221243,#221244,#221245,#221246,#221247,#221248,#221249,#221250,#221251,
#221252,#221253,#221254,#221255,#221256,#221257,#221258,#221259,#221260,
#221261,#221262,#221263,#221264,#221265,#221266,#221267,#221268),
 .UNSPECIFIED.,.F.,.F.,(4,3,3,3,3,3,3,3,3,3,3,3,3,4),(0.,6.80370855342904E-5,
0.000137303169293723,0.000203636706656155,0.000256396220959708,0.000256540237295735,
0.000285209320207743,0.000342105100635661,0.0003847769359566,0.000400778874201952,
0.000456785658060683,0.000484789049990049,0.000498790745954732,0.000512792441919415),
 .UNSPECIFIED.);
#4973=B_SPLINE_CURVE_WITH_KNOTS('',3,(#221272,#221273,#221274,#221275,#221276,
#221277,#221278,#221279,#221280,#221281,#221282,#221283,#221284,#221285,
#221286,#221287,#221288,#221289,#221290,#221291,#221292,#221293,#221294,
#221295,#221296,#221297,#221298,#221299,#221300,#221301,#221302,#221303,
#221304,#221305,#221306,#221307,#221308),.UNSPECIFIED.,.F.,.F.,(4,3,3,3,
3,3,3,3,3,3,3,3,4),(0.,1.12535551670994E-5,7.76936938473578E-5,0.000102513517961135,
0.000121879189824281,0.000189659041345291,0.000223548967105796,0.000257294099096098,
0.000257438892866302,0.000325720851756026,0.000396486773956574,0.000466242707664513,
0.000514877785732603),.UNSPECIFIED.);
#4974=B_SPLINE_CURVE_WITH_KNOTS('',3,(#221315,#221316,#221317,#221318,#221319,
#221320,#221321,#221322,#221323,#221324,#221325,#221326,#221327,#221328,
#221329,#221330,#221331,#221332,#221333,#221334,#221335,#221336,#221337,
#221338,#221339,#221340,#221341,#221342,#221343,#221344,#221345,#221346,
#221347,#221348,#221349,#221350,#221351,#221352,#221353,#221354),
 .UNSPECIFIED.,.F.,.F.,(4,3,3,3,3,3,3,3,3,3,3,3,3,4),(0.,6.80370855359559E-5,
0.000137303169297146,0.000203636706661351,0.000256396220959708,0.000256540237295741,
0.000285209320207738,0.000342105100635657,0.000384776935956596,0.000400778874201949,
0.000456785658060682,0.000484789049990049,0.000498790745954732,0.000512792441919415),
 .UNSPECIFIED.);
#4975=B_SPLINE_CURVE_WITH_KNOTS('',3,(#224968,#224969,#224970,#224971,#224972,
#224973,#224974,#224975,#224976,#224977,#224978,#224979,#224980,#224981,
#224982,#224983,#224984,#224985,#224986,#224987,#224988,#224989,#224990,
#224991,#224992,#224993,#224994,#224995,#224996,#224997,#224998,#224999,
#225000,#225001,#225002,#225003,#225004,#225005,#225006,#225007,#225008,
#225009,#225010,#225011,#225012,#225013,#225014,#225015,#225016,#225017,
#225018,#225019),.UNSPECIFIED.,.F.,.F.,(4,3,3,3,3,3,3,3,3,3,3,3,3,3,3,3,
3,4),(0.,4.30706237870626E-5,8.47417087698098E-5,0.000124159989205863,0.000160467076290102,
0.000170998382116694,0.000182414994733773,0.000213747977645868,0.000242415955903168,
0.000256497573175041,0.000259169422895615,0.00026175777731242,0.00028996513040335,
0.000301877270772904,0.000321937017503146,0.000326951954185707,0.000334474359209548,
0.000341996764233388),.UNSPECIFIED.);
#4976=B_SPLINE_CURVE_WITH_KNOTS('',3,(#225020,#225021,#225022,#225023,#225024,
#225025,#225026,#225027,#225028,#225029,#225030,#225031,#225032,#225033,
#225034,#225035,#225036,#225037,#225038,#225039,#225040,#225041,#225042,
#225043,#225044,#225045,#225046,#225047,#225048,#225049,#225050,#225051,
#225052,#225053,#225054,#225055,#225056,#225057,#225058,#225059,#225060,
#225061,#225062,#225063,#225064,#225065,#225066,#225067,#225068,#225069,
#225070,#225071),.UNSPECIFIED.,.F.,.F.,(4,3,3,3,3,3,3,3,3,3,3,3,3,3,3,3,
3,4),(0.,2.58457451675679E-5,4.2539444619485E-5,6.46659869686642E-5,7.57292581432538E-5,
8.12608937305486E-5,8.26438026273723E-5,8.67925293178434E-5,0.000116015624426966,
0.000130188793976765,0.000151886926306226,0.00016196365121128,0.000162735992470956,
0.000173585058635687,0.000212487880461617,0.000255238173514508,0.000301397761155089,
0.000347170117271359),.UNSPECIFIED.);
#4977=B_SPLINE_CURVE_WITH_KNOTS('',3,(#225073,#225074,#225075,#225076,#225077,
#225078,#225079,#225080,#225081,#225082,#225083,#225084,#225085,#225086,
#225087,#225088,#225089,#225090,#225091,#225092,#225093,#225094,#225095,
#225096,#225097,#225098,#225099,#225100,#225101,#225102,#225103,#225104,
#225105,#225106,#225107,#225108,#225109,#225110,#225111,#225112,#225113,
#225114,#225115,#225116,#225117,#225118),.UNSPECIFIED.,.F.,.F.,(4,3,3,3,
3,3,3,3,3,3,3,3,3,3,3,4),(3.3881317890172E-21,2.57218161987639E-5,4.21568322569294E-5,
6.4587331461773E-5,7.58025810641948E-5,8.14102058654057E-5,8.28121120657085E-5,
8.70178306666167E-5,0.000116081955658157,0.000130526745999925,0.000162394111022045,
0.000174035661333233,0.000213138396957335,0.000256116935431967,0.000302406662853213,
0.000348071322666466),.UNSPECIFIED.);
#4978=B_SPLINE_CURVE_WITH_KNOTS('',3,(#225119,#225120,#225121,#225122,#225123,
#225124,#225125,#225126,#225127,#225128,#225129,#225130,#225131,#225132,
#225133,#225134,#225135,#225136,#225137,#225138,#225139,#225140,#225141,
#225142,#225143,#225144,#225145,#225146,#225147,#225148,#225149,#225150,
#225151,#225152,#225153,#225154,#225155,#225156,#225157,#225158,#225159,
#225160,#225161,#225162,#225163,#225164,#225165,#225166,#225167,#225168,
#225169,#225170),.UNSPECIFIED.,.F.,.F.,(4,3,3,3,3,3,3,3,3,3,3,3,3,3,3,3,
3,4),(0.,4.29652152146413E-5,8.44519107510641E-5,0.000123669830862078,0.000159788877354881,
0.000170558847912631,0.000181218775907171,0.000181960046452396,0.000214460062643458,
0.000244755726198141,0.000255838271868947,0.000258503253867582,0.000261084955178759,
0.000289370476647919,0.000301101325502011,0.000321109510663637,0.00033111360324445,
0.000341117695825263),.UNSPECIFIED.);
#4979=B_SPLINE_CURVE_WITH_KNOTS('',3,(#228853,#228854,#228855,#228856,#228857,
#228858,#228859,#228860,#228861,#228862,#228863,#228864,#228865,#228866,
#228867,#228868,#228869,#228870,#228871,#228872,#228873,#228874,#228875,
#228876,#228877,#228878,#228879,#228880,#228881,#228882,#228883,#228884,
#228885,#228886,#228887,#228888,#228889,#228890,#228891,#228892,#228893,
#228894,#228895,#228896,#228897,#228898,#228899,#228900,#228901,#228902,
#228903,#228904),.UNSPECIFIED.,.F.,.F.,(4,3,3,3,3,3,3,3,3,3,3,3,3,3,3,3,
3,4),(0.,4.30706237887532E-5,8.4741708772828E-5,0.000124159989210102,0.000160467076295626,
0.000170998382116695,0.000182414994733766,0.000213747977645869,0.000242415955903966,
0.000256497573175043,0.000259169422895616,0.000261757777312422,0.000289965130402892,
0.000301877270772906,0.000321937017503149,0.000326951954185709,0.00033447435920955,
0.000341996764233391),.UNSPECIFIED.);
#4980=B_SPLINE_CURVE_WITH_KNOTS('',3,(#228905,#228906,#228907,#228908,#228909,
#228910,#228911,#228912,#228913,#228914,#228915,#228916,#228917,#228918,
#228919,#228920,#228921,#228922,#228923,#228924,#228925,#228926,#228927,
#228928,#228929,#228930,#228931,#228932,#228933,#228934,#228935,#228936,
#228937,#228938,#228939,#228940,#228941,#228942,#228943,#228944,#228945,
#228946,#228947,#228948,#228949,#228950,#228951,#228952,#228953,#228954,
#228955,#228956),.UNSPECIFIED.,.F.,.F.,(4,3,3,3,3,3,3,3,3,3,3,3,3,3,3,3,
3,4),(8.67361737988404E-19,2.58457451673786E-5,4.25394446195963E-5,6.4665986968718E-5,
7.57292581432788E-5,8.12608937305592E-5,8.26438026273793E-5,8.67925293178396E-5,
0.000116015624426922,0.000130188793976759,0.000151886926306219,0.000161963651211269,
0.000162735992470948,0.000173585058635678,0.000212487880462208,0.000255238173514594,
0.000301397761152511,0.000347170117271357),.UNSPECIFIED.);
#4981=B_SPLINE_CURVE_WITH_KNOTS('',3,(#228958,#228959,#228960,#228961,#228962,
#228963,#228964,#228965,#228966,#228967,#228968,#228969,#228970,#228971,
#228972,#228973,#228974,#228975,#228976,#228977,#228978,#228979,#228980,
#228981,#228982,#228983,#228984,#228985,#228986,#228987,#228988,#228989,
#228990,#228991,#228992,#228993,#228994,#228995,#228996,#228997,#228998,
#228999,#229000,#229001,#229002,#229003),.UNSPECIFIED.,.F.,.F.,(4,3,3,3,
3,3,3,3,3,3,3,3,3,3,3,4),(0.,2.57218162000954E-5,4.21568322569208E-5,6.45873314617704E-5,
7.58025810641952E-5,8.14102058654076E-5,8.28121120657107E-5,8.701783066662E-5,
0.000116081955658867,0.000130526745999926,0.000162394111022053,0.000174035661333232,
0.000213138396959432,0.000256116935436117,0.000302406662859553,0.00034807132266647),
 .UNSPECIFIED.);
#4982=B_SPLINE_CURVE_WITH_KNOTS('',3,(#229004,#229005,#229006,#229007,#229008,
#229009,#229010,#229011,#229012,#229013,#229014,#229015,#229016,#229017,
#229018,#229019,#229020,#229021,#229022,#229023,#229024,#229025,#229026,
#229027,#229028,#229029,#229030,#229031,#229032,#229033,#229034,#229035,
#229036,#229037,#229038,#229039,#229040,#229041,#229042,#229043,#229044,
#229045,#229046,#229047,#229048,#229049,#229050,#229051,#229052,#229053,
#229054,#229055),.UNSPECIFIED.,.F.,.F.,(4,3,3,3,3,3,3,3,3,3,3,3,3,3,3,3,
3,4),(0.,4.29652152129061E-5,8.44519107484223E-5,0.000123669830859236,0.000159788877352066,
0.000170558847912624,0.000181218775907164,0.000181960046452401,0.000214460062644132,
0.000244755726200044,0.000255838271868943,0.000258503253867578,0.000261084955178755,
0.000289370476646873,0.000301101325502008,0.000321109510663635,0.000331113603244448,
0.000341117695825261),.UNSPECIFIED.);
#4983=B_SPLINE_CURVE_WITH_KNOTS('',3,(#229057,#229058,#229059,#229060,#229061,
#229062,#229063,#229064,#229065,#229066,#229067,#229068,#229069,#229070,
#229071,#229072,#229073,#229074,#229075,#229076,#229077,#229078,#229079,
#229080,#229081,#229082,#229083,#229084,#229085,#229086,#229087,#229088,
#229089,#229090,#229091,#229092,#229093,#229094,#229095,#229096,#229097,
#229098,#229099,#229100,#229101,#229102,#229103,#229104,#229105,#229106,
#229107,#229108),.UNSPECIFIED.,.F.,.F.,(4,3,3,3,3,3,3,3,3,3,3,3,3,3,3,3,
3,4),(0.,4.30706237867375E-5,8.47417087691522E-5,0.000124159989204823,0.00016046707628857,
0.000170998382116696,0.000182414994733785,0.000213747977645869,0.000242415955903806,
0.000256497573175043,0.000259169422895616,0.000261757777312422,0.000289965130402222,
0.000301877270772906,0.000321937017503148,0.000326951954185709,0.00033447435920955,
0.00034199676423339),.UNSPECIFIED.);
#4984=B_SPLINE_CURVE_WITH_KNOTS('',3,(#229109,#229110,#229111,#229112,#229113,
#229114,#229115,#229116,#229117,#229118,#229119,#229120,#229121,#229122,
#229123,#229124,#229125,#229126,#229127,#229128,#229129,#229130,#229131,
#229132,#229133,#229134,#229135,#229136,#229137,#229138,#229139,#229140,
#229141,#229142,#229143,#229144,#229145,#229146,#229147,#229148,#229149,
#229150,#229151,#229152,#229153,#229154,#229155,#229156,#229157,#229158,
#229159,#229160),.UNSPECIFIED.,.F.,.F.,(4,3,3,3,3,3,3,3,3,3,3,3,3,3,3,3,
3,4),(0.,2.58457451687563E-5,4.25394446196343E-5,6.46659869687391E-5,7.57292581432915E-5,
8.12608937305677E-5,8.26438026273867E-5,8.67925293178438E-5,0.000116015624427484,
0.000130188793976766,0.000151886926306227,0.000161963651211279,0.000162735992470957,
0.000173585058635688,0.000212487880458173,0.000255238173505986,0.000301397761137943,
0.000347170117271372),.UNSPECIFIED.);
#4985=B_SPLINE_CURVE_WITH_KNOTS('',3,(#229162,#229163,#229164,#229165,#229166,
#229167,#229168,#229169,#229170,#229171,#229172,#229173,#229174,#229175,
#229176,#229177,#229178,#229179,#229180,#229181,#229182,#229183,#229184,
#229185,#229186,#229187,#229188,#229189,#229190,#229191,#229192,#229193,
#229194,#229195,#229196,#229197,#229198,#229199,#229200,#229201,#229202,
#229203,#229204,#229205,#229206,#229207),.UNSPECIFIED.,.F.,.F.,(4,3,3,3,
3,3,3,3,3,3,3,3,3,3,3,4),(1.73472347597681E-18,2.57218161994071E-5,4.21568322567322E-5,
6.45873314616717E-5,7.58025810641414E-5,8.14102058653763E-5,8.2812112065685E-5,
8.70178306666112E-5,0.000116081955658581,0.000130526745999916,0.000162394111022036,
0.000174035661333221,0.000213138396957988,0.00025611693543334,0.000302406662855556,
0.000348071322666432),.UNSPECIFIED.);
#4986=B_SPLINE_CURVE_WITH_KNOTS('',3,(#229208,#229209,#229210,#229211,#229212,
#229213,#229214,#229215,#229216,#229217,#229218,#229219,#229220,#229221,
#229222,#229223,#229224,#229225,#229226,#229227,#229228,#229229,#229230,
#229231,#229232,#229233,#229234,#229235,#229236,#229237,#229238,#229239,
#229240,#229241,#229242,#229243,#229244,#229245,#229246,#229247,#229248,
#229249,#229250,#229251,#229252,#229253,#229254,#229255,#229256,#229257,
#229258,#229259),.UNSPECIFIED.,.F.,.F.,(4,3,3,3,3,3,3,3,3,3,3,3,3,3,3,3,
3,4),(0.,4.2965215217082E-5,8.44519107547709E-5,0.000123669830866139,0.00015978887735852,
0.000170558847912625,0.000181218775907164,0.00018196004645241,0.000214460062644103,
0.000244755726200267,0.000255838271868937,0.000258503253867572,0.000261084955178749,
0.000289370476647232,0.000301101325501999,0.000321109510663624,0.000331113603244437,
0.000341117695825249),.UNSPECIFIED.);
#4987=B_SPLINE_CURVE_WITH_KNOTS('',3,(#229261,#229262,#229263,#229264,#229265,
#229266,#229267,#229268,#229269,#229270,#229271,#229272,#229273,#229274,
#229275,#229276,#229277,#229278,#229279,#229280,#229281,#229282,#229283,
#229284,#229285,#229286,#229287,#229288,#229289,#229290,#229291,#229292,
#229293,#229294,#229295,#229296,#229297,#229298,#229299,#229300,#229301,
#229302,#229303,#229304,#229305,#229306,#229307,#229308,#229309,#229310,
#229311,#229312),.UNSPECIFIED.,.F.,.F.,(4,3,3,3,3,3,3,3,3,3,3,3,3,3,3,3,
3,4),(9.81307786677359E-18,4.30706237882728E-5,8.4741708772019E-5,0.000124159989209085,
0.000160467076294421,0.000170998382116706,0.000182414994733799,0.000213747977645876,
0.000242415955904087,0.000256497573175047,0.00025916942289562,0.000261757777312426,
0.000289965130402721,0.000301877270772907,0.000321937017503148,0.000326951954185708,
0.000334474359209548,0.000341996764233389),.UNSPECIFIED.);
#4988=B_SPLINE_CURVE_WITH_KNOTS('',3,(#229313,#229314,#229315,#229316,#229317,
#229318,#229319,#229320,#229321,#229322,#229323,#229324,#229325,#229326,
#229327,#229328,#229329,#229330,#229331,#229332,#229333,#229334,#229335,
#229336,#229337,#229338,#229339,#229340,#229341,#229342,#229343,#229344,
#229345,#229346,#229347,#229348,#229349,#229350,#229351,#229352,#229353,
#229354,#229355,#229356,#229357,#229358,#229359,#229360,#229361,#229362,
#229363,#229364),.UNSPECIFIED.,.F.,.F.,(4,3,3,3,3,3,3,3,3,3,3,3,3,3,3,3,
3,4),(0.,2.58457451680732E-5,4.25394446195484E-5,6.46659869686971E-5,7.57292581432714E-5,
8.12608937305585E-5,8.26438026273803E-5,8.67925293178457E-5,0.000116015624427878,
0.000130188793976769,0.00015188692630623,0.000161963651211275,0.000162735992470961,
0.000173585058635691,0.000212487880461201,0.000255238173511369,0.000301397761144767,
0.000347170117271375),.UNSPECIFIED.);
#4989=B_SPLINE_CURVE_WITH_KNOTS('',3,(#229366,#229367,#229368,#229369,#229370,
#229371,#229372,#229373,#229374,#229375,#229376,#229377,#229378,#229379,
#229380,#229381,#229382,#229383,#229384,#229385,#229386,#229387,#229388,
#229389,#229390,#229391,#229392,#229393,#229394,#229395,#229396,#229397,
#229398,#229399,#229400,#229401,#229402,#229403,#229404,#229405,#229406,
#229407,#229408,#229409,#229410,#229411),.UNSPECIFIED.,.F.,.F.,(4,3,3,3,
3,3,3,3,3,3,3,3,3,3,3,4),(0.,2.57218161998569E-5,4.21568322567428E-5,6.45873314616809E-5,
7.580258106415E-5,8.14102058653845E-5,8.28121120656931E-5,8.7017830666619E-5,
0.000116081955658763,0.000130526745999929,0.000162394111022056,0.000174035661333238,
0.000213138396959539,0.000256116935436271,0.000302406662859608,0.000348071322666466),
 .UNSPECIFIED.);
#4990=B_SPLINE_CURVE_WITH_KNOTS('',3,(#229412,#229413,#229414,#229415,#229416,
#229417,#229418,#229419,#229420,#229421,#229422,#229423,#229424,#229425,
#229426,#229427,#229428,#229429,#229430,#229431,#229432,#229433,#229434,
#229435,#229436,#229437,#229438,#229439,#229440,#229441,#229442,#229443,
#229444,#229445,#229446,#229447,#229448,#229449,#229450,#229451,#229452,
#229453,#229454,#229455,#229456,#229457,#229458,#229459,#229460,#229461,
#229462,#229463),.UNSPECIFIED.,.F.,.F.,(4,3,3,3,3,3,3,3,3,3,3,3,3,3,3,3,
3,4),(4.33680868994202E-19,4.29652152167429E-5,8.44519107544172E-5,0.00012366983086611,
0.000159788877359186,0.000170558847912624,0.000181218775907164,0.000181960046452399,
0.000214460062644025,0.000244755726199709,0.000255838271868944,0.000258503253867579,
0.000261084955178756,0.000289370476647272,0.00030110132550201,0.000321109510663636,
0.00033111360324445,0.000341117695825263),.UNSPECIFIED.);
#4991=B_SPLINE_CURVE_WITH_KNOTS('',3,(#229465,#229466,#229467,#229468,#229469,
#229470,#229471,#229472,#229473,#229474,#229475,#229476,#229477,#229478,
#229479,#229480,#229481,#229482,#229483,#229484,#229485,#229486,#229487,
#229488,#229489,#229490,#229491,#229492,#229493,#229494,#229495,#229496,
#229497,#229498,#229499,#229500,#229501,#229502,#229503,#229504,#229505,
#229506,#229507,#229508,#229509,#229510,#229511,#229512,#229513,#229514,
#229515,#229516),.UNSPECIFIED.,.F.,.F.,(4,3,3,3,3,3,3,3,3,3,3,3,3,3,3,3,
3,4),(0.,4.30706237880298E-5,8.47417087716239E-5,0.000124159989208614,0.000160467076293979,
0.000170998382116694,0.00018241499473377,0.000213747977645868,0.000242415955903985,
0.000256497573175042,0.000259169422895615,0.00026175777731242,0.00028996513040211,
0.000301877270772905,0.000321937017503147,0.000326951954185707,0.000334474359209548,
0.000341996764233389),.UNSPECIFIED.);
#4992=B_SPLINE_CURVE_WITH_KNOTS('',3,(#229517,#229518,#229519,#229520,#229521,
#229522,#229523,#229524,#229525,#229526,#229527,#229528,#229529,#229530,
#229531,#229532,#229533,#229534,#229535,#229536,#229537,#229538,#229539,
#229540,#229541,#229542,#229543,#229544,#229545,#229546,#229547,#229548,
#229549,#229550,#229551,#229552,#229553,#229554,#229555,#229556,#229557,
#229558,#229559,#229560,#229561,#229562,#229563,#229564,#229565,#229566,
#229567,#229568),.UNSPECIFIED.,.F.,.F.,(4,3,3,3,3,3,3,3,3,3,3,3,3,3,3,3,
3,4),(0.,2.58457451667647E-5,4.25394446195672E-5,6.46659869687037E-5,7.57292581432719E-5,
8.1260893730556E-5,8.2643802627377E-5,8.67925293178401E-5,0.000116015624426914,
0.00013018879397676,0.00015188692630622,0.000161963651211274,0.00016273599247095,
0.00017358505863568,0.000212487880460383,0.000255238173510125,0.000301397761143776,
0.000347170117271361),.UNSPECIFIED.);
#4993=B_SPLINE_CURVE_WITH_KNOTS('',3,(#229570,#229571,#229572,#229573,#229574,
#229575,#229576,#229577,#229578,#229579,#229580,#229581,#229582,#229583,
#229584,#229585,#229586,#229587,#229588,#229589,#229590,#229591,#229592,
#229593,#229594,#229595,#229596,#229597,#229598,#229599,#229600,#229601,
#229602,#229603,#229604,#229605,#229606,#229607,#229608,#229609,#229610,
#229611,#229612,#229613,#229614,#229615),.UNSPECIFIED.,.F.,.F.,(4,3,3,3,
3,3,3,3,3,3,3,3,3,3,3,4),(3.46944695195361E-18,2.57218161985872E-5,4.21568322569015E-5,
6.458733146176E-5,7.58025810641893E-5,8.14102058654039E-5,8.28121120657076E-5,
8.70178306666186E-5,0.000116081955658227,0.000130526745999926,0.000162394111022037,
0.000174035661333234,0.000213138396958737,0.000256116935434941,0.000302406662858469,
0.000348071322666472),.UNSPECIFIED.);
#4994=B_SPLINE_CURVE_WITH_KNOTS('',3,(#229616,#229617,#229618,#229619,#229620,
#229621,#229622,#229623,#229624,#229625,#229626,#229627,#229628,#229629,
#229630,#229631,#229632,#229633,#229634,#229635,#229636,#229637,#229638,
#229639,#229640,#229641,#229642,#229643,#229644,#229645,#229646,#229647,
#229648,#229649,#229650,#229651,#229652,#229653,#229654,#229655,#229656,
#229657,#229658,#229659,#229660,#229661,#229662,#229663,#229664,#229665,
#229666,#229667),.UNSPECIFIED.,.F.,.F.,(4,3,3,3,3,3,3,3,3,3,3,3,3,3,3,3,
3,4),(0.,4.29652152154219E-5,8.44519107522863E-5,0.000123669830863478,0.000159788877356216,
0.000170558847912624,0.000181218775907164,0.000181960046452393,0.000214460062643201,
0.000244755726197205,0.000255838271868943,0.000258503253867578,0.000261084955178756,
0.000289370476648893,0.00030110132550201,0.000321109510663636,0.00033111360324445,
0.000341117695825263),.UNSPECIFIED.);
#4995=B_SPLINE_CURVE_WITH_KNOTS('',3,(#229669,#229670,#229671,#229672,#229673,
#229674,#229675,#229676,#229677,#229678,#229679,#229680,#229681,#229682,
#229683,#229684,#229685,#229686,#229687,#229688,#229689,#229690,#229691,
#229692,#229693,#229694,#229695,#229696,#229697,#229698,#229699,#229700,
#229701,#229702,#229703,#229704,#229705,#229706,#229707,#229708,#229709,
#229710,#229711,#229712,#229713,#229714,#229715,#229716,#229717,#229718,
#229719,#229720),.UNSPECIFIED.,.F.,.F.,(4,3,3,3,3,3,3,3,3,3,3,3,3,3,3,3,
3,4),(0.,4.30706237873536E-5,8.47417087703233E-5,0.000124159989206582,0.000160467076290998,
0.000170998382116696,0.00018241499473377,0.000213747977645869,0.000242415955903727,
0.000256497573175043,0.000259169422895616,0.000261757777312422,0.000289965130402594,
0.000301877270772906,0.000321937017503148,0.000326951954185709,0.00033447435920955,
0.000341996764233391),.UNSPECIFIED.);
#4996=B_SPLINE_CURVE_WITH_KNOTS('',3,(#229721,#229722,#229723,#229724,#229725,
#229726,#229727,#229728,#229729,#229730,#229731,#229732,#229733,#229734,
#229735,#229736,#229737,#229738,#229739,#229740,#229741,#229742,#229743,
#229744,#229745,#229746,#229747,#229748,#229749,#229750,#229751,#229752,
#229753,#229754,#229755,#229756,#229757,#229758,#229759,#229760,#229761,
#229762,#229763,#229764,#229765,#229766,#229767,#229768,#229769,#229770,
#229771,#229772),.UNSPECIFIED.,.F.,.F.,(4,3,3,3,3,3,3,3,3,3,3,3,3,3,3,3,
3,4),(3.46944695195361E-18,2.58457451679116E-5,4.25394446195865E-5,6.46659869687166E-5,
7.57292581432817E-5,8.12608937305642E-5,8.26438026273848E-5,8.67925293178467E-5,
0.000116015624426944,0.000130188793976768,0.000151886926306229,0.00016196365121128,
0.00016273599247096,0.00017358505863569,0.000212487880461716,0.000255238173512545,
0.000301397761146856,0.000347170117271378),.UNSPECIFIED.);
#4997=B_SPLINE_CURVE_WITH_KNOTS('',3,(#229774,#229775,#229776,#229777,#229778,
#229779,#229780,#229781,#229782,#229783,#229784,#229785,#229786,#229787,
#229788,#229789,#229790,#229791,#229792,#229793,#229794,#229795,#229796,
#229797,#229798,#229799,#229800,#229801,#229802,#229803,#229804,#229805,
#229806,#229807,#229808,#229809,#229810,#229811,#229812,#229813,#229814,
#229815,#229816,#229817,#229818,#229819),.UNSPECIFIED.,.F.,.F.,(4,3,3,3,
3,3,3,3,3,3,3,3,3,3,3,4),(0.,2.5721816201399E-5,4.21568322568262E-5,6.45873314617204E-5,
7.58025810641675E-5,8.14102058653911E-5,8.28121120656969E-5,8.70178306666146E-5,
0.000116081955658794,0.000130526745999922,0.00016239411102205,0.000174035661333229,
0.000213138396959652,0.000256116935436567,0.000302406662860262,0.000348071322666458),
 .UNSPECIFIED.);
#4998=B_SPLINE_CURVE_WITH_KNOTS('',3,(#229820,#229821,#229822,#229823,#229824,
#229825,#229826,#229827,#229828,#229829,#229830,#229831,#229832,#229833,
#229834,#229835,#229836,#229837,#229838,#229839,#229840,#229841,#229842,
#229843,#229844,#229845,#229846,#229847,#229848,#229849,#229850,#229851,
#229852,#229853,#229854,#229855,#229856,#229857,#229858,#229859,#229860,
#229861,#229862,#229863,#229864,#229865,#229866,#229867,#229868,#229869,
#229870,#229871),.UNSPECIFIED.,.F.,.F.,(4,3,3,3,3,3,3,3,3,3,3,3,3,3,3,3,
3,4),(1.30104260698261E-18,4.29652152181542E-5,8.44519107567955E-5,0.000123669830869214,
0.000159788877362927,0.000170558847912638,0.000181218775907177,0.000181960046452419,
0.000214460062643728,0.000244755726198606,0.000255838271868948,0.000258503253867583,
0.00026108495517876,0.000289370476648016,0.000301101325502009,0.000321109510663634,
0.000331113603244446,0.000341117695825258),.UNSPECIFIED.);
#4999=B_SPLINE_CURVE_WITH_KNOTS('',3,(#229873,#229874,#229875,#229876,#229877,
#229878,#229879,#229880,#229881,#229882,#229883,#229884,#229885,#229886,
#229887,#229888,#229889,#229890,#229891,#229892,#229893,#229894,#229895,
#229896,#229897,#229898,#229899,#229900,#229901,#229902,#229903,#229904,
#229905,#229906,#229907,#229908,#229909,#229910,#229911,#229912,#229913,
#229914,#229915,#229916,#229917,#229918,#229919,#229920,#229921,#229922,
#229923,#229924),.UNSPECIFIED.,.F.,.F.,(4,3,3,3,3,3,3,3,3,3,3,3,3,3,3,3,
3,4),(1.25393031850254E-17,4.30706237863908E-5,8.47417087685059E-5,0.000124159989203962,
0.000160467076287454,0.000170998382116688,0.000182414994733768,0.000213747977645861,
0.000242415955902704,0.000256497573175034,0.000259169422895607,0.000261757777312413,
0.000289965130403529,0.000301877270772897,0.000321937017503139,0.000326951954185699,
0.00033447435920954,0.000341996764233381),.UNSPECIFIED.);
#5000=B_SPLINE_CURVE_WITH_KNOTS('',3,(#229925,#229926,#229927,#229928,#229929,
#229930,#229931,#229932,#229933,#229934,#229935,#229936,#229937,#229938,
#229939,#229940,#229941,#229942,#229943,#229944,#229945,#229946,#229947,
#229948,#229949,#229950,#229951,#229952,#229953,#229954,#229955,#229956,
#229957,#229958,#229959,#229960,#229961,#229962,#229963,#229964,#229965,
#229966,#229967,#229968,#229969,#229970,#229971,#229972,#229973,#229974,
#229975,#229976),.UNSPECIFIED.,.F.,.F.,(4,3,3,3,3,3,3,3,3,3,3,3,3,3,3,3,
3,4),(0.,2.58457451685014E-5,4.2539444619537E-5,6.4665986968689E-5,7.57292581432651E-5,
8.12608937305531E-5,8.26438026273751E-5,8.67925293178411E-5,0.000116015624427711,
0.000130188793976762,0.000151886926306222,0.000161963651211274,0.000162735992470952,
0.000173585058635682,0.000212487880459268,0.000255238173508192,0.000301397761141237,
0.000347170117271364),.UNSPECIFIED.);
#5001=B_SPLINE_CURVE_WITH_KNOTS('',3,(#229978,#229979,#229980,#229981,#229982,
#229983,#229984,#229985,#229986,#229987,#229988,#229989,#229990,#229991,
#229992,#229993,#229994,#229995,#229996,#229997,#229998,#229999,#230000,
#230001,#230002,#230003,#230004,#230005,#230006,#230007,#230008,#230009,
#230010,#230011,#230012,#230013,#230014,#230015,#230016,#230017,#230018,
#230019,#230020,#230021,#230022,#230023),.UNSPECIFIED.,.F.,.F.,(4,3,3,3,
3,3,3,3,3,3,3,3,3,3,3,4),(0.,2.5721816199478E-5,4.21568322567195E-5,6.45873314616702E-5,
7.58025810641455E-5,8.14102058653832E-5,8.28121120656926E-5,8.70178306666208E-5,
0.000116081955658429,0.000130526745999931,0.000162394111022058,0.000174035661333242,
0.000213138396959934,0.000256116935437069,0.000302406662860884,0.000348071322666478),
 .UNSPECIFIED.);
#5002=B_SPLINE_CURVE_WITH_KNOTS('',3,(#230024,#230025,#230026,#230027,#230028,
#230029,#230030,#230031,#230032,#230033,#230034,#230035,#230036,#230037,
#230038,#230039,#230040,#230041,#230042,#230043,#230044,#230045,#230046,
#230047,#230048,#230049,#230050,#230051,#230052,#230053,#230054,#230055,
#230056,#230057,#230058,#230059,#230060,#230061,#230062,#230063,#230064,
#230065,#230066,#230067,#230068,#230069,#230070,#230071,#230072,#230073,
#230074,#230075),.UNSPECIFIED.,.F.,.F.,(4,3,3,3,3,3,3,3,3,3,3,3,3,3,3,3,
3,4),(1.73472347597681E-18,4.29652152148517E-5,8.44519107515775E-5,0.000123669830863035,
0.000159788877356324,0.000170558847912634,0.000181218775907174,0.000181960046452412,
0.000214460062643518,0.000244755726197894,0.000255838271868951,0.000258503253867585,
0.000261084955178763,0.000289370476647261,0.000301101325502015,0.000321109510663641,
0.000331113603244454,0.000341117695825267),.UNSPECIFIED.);
#5003=B_SPLINE_CURVE_WITH_KNOTS('',3,(#230077,#230078,#230079,#230080,#230081,
#230082,#230083,#230084,#230085,#230086,#230087,#230088,#230089,#230090,
#230091,#230092,#230093,#230094,#230095,#230096,#230097,#230098,#230099,
#230100,#230101,#230102,#230103,#230104,#230105,#230106,#230107,#230108,
#230109,#230110,#230111,#230112,#230113,#230114,#230115,#230116,#230117,
#230118,#230119,#230120,#230121,#230122,#230123,#230124,#230125,#230126,
#230127,#230128),.UNSPECIFIED.,.F.,.F.,(4,3,3,3,3,3,3,3,3,3,3,3,3,3,3,3,
3,4),(0.,4.30706237876963E-5,8.47417087710402E-5,0.000124159989207774,0.000160467076292755,
0.000170998382116703,0.000182414994733789,0.000213747977645875,0.000242415955903658,
0.000256497573175047,0.00025916942289562,0.000261757777312425,0.0002899651304043,
0.000301877270772908,0.000321937017503149,0.000326951954185709,0.00033447435920955,
0.00034199676423339),.UNSPECIFIED.);
#5004=B_SPLINE_CURVE_WITH_KNOTS('',3,(#230129,#230130,#230131,#230132,#230133,
#230134,#230135,#230136,#230137,#230138,#230139,#230140,#230141,#230142,
#230143,#230144,#230145,#230146,#230147,#230148,#230149,#230150,#230151,
#230152,#230153,#230154,#230155,#230156,#230157,#230158,#230159,#230160,
#230161,#230162,#230163,#230164,#230165,#230166,#230167,#230168,#230169,
#230170,#230171,#230172,#230173,#230174,#230175,#230176,#230177,#230178,
#230179,#230180),.UNSPECIFIED.,.F.,.F.,(4,3,3,3,3,3,3,3,3,3,3,3,3,3,3,3,
3,4),(0.,2.58457451675268E-5,4.2539444619566E-5,6.46659869687072E-5,7.57292581432777E-5,
8.1260893730563E-5,8.26438026273844E-5,8.67925293178483E-5,0.000116015624427071,
0.000130188793976773,0.000151886926306235,0.000161963651211294,0.000162735992470966,
0.000173585058635697,0.000212487880460834,0.000255238173511205,0.000301397761145922,
0.000347170117271376),.UNSPECIFIED.);
#5005=B_SPLINE_CURVE_WITH_KNOTS('',3,(#230182,#230183,#230184,#230185,#230186,
#230187,#230188,#230189,#230190,#230191,#230192,#230193,#230194,#230195,
#230196,#230197,#230198,#230199,#230200,#230201,#230202,#230203,#230204,
#230205,#230206,#230207,#230208,#230209,#230210,#230211,#230212,#230213,
#230214,#230215,#230216,#230217,#230218,#230219,#230220,#230221,#230222,
#230223,#230224,#230225,#230226,#230227),.UNSPECIFIED.,.F.,.F.,(4,3,3,3,
3,3,3,3,3,3,3,3,3,3,3,4),(0.,2.57218161991606E-5,4.21568322569619E-5,6.45873314617843E-5,
7.58025810641956E-5,8.14102058654012E-5,8.28121120657026E-5,8.70178306666068E-5,
0.000116081955658637,0.00013052674599991,0.000162394111022018,0.000174035661333214,
0.000213138396962703,0.00025611693544274,0.000302406662870117,0.000348071322666447),
 .UNSPECIFIED.);
#5006=B_SPLINE_CURVE_WITH_KNOTS('',3,(#230228,#230229,#230230,#230231,#230232,
#230233,#230234,#230235,#230236,#230237,#230238,#230239,#230240,#230241,
#230242,#230243,#230244,#230245,#230246,#230247,#230248,#230249,#230250,
#230251,#230252,#230253,#230254,#230255,#230256,#230257,#230258,#230259,
#230260,#230261,#230262,#230263,#230264,#230265,#230266,#230267,#230268,
#230269,#230270,#230271,#230272,#230273,#230274,#230275,#230276,#230277,
#230278,#230279),.UNSPECIFIED.,.F.,.F.,(4,3,3,3,3,3,3,3,3,3,3,3,3,3,3,3,
3,4),(1.30104260698261E-18,4.2965215217907E-5,8.44519107568489E-5,0.000123669830870173,
0.000159788877365401,0.000170558847912636,0.000181218775907176,0.000181960046452404,
0.000214460062644115,0.000244755726199935,0.000255838271868953,0.000258503253867588,
0.000261084955178766,0.000289370476646324,0.000301101325502018,0.000321109510663644,
0.000331113603244457,0.00034111769582527),.UNSPECIFIED.);
#5007=B_SPLINE_CURVE_WITH_KNOTS('',3,(#230281,#230282,#230283,#230284,#230285,
#230286,#230287,#230288,#230289,#230290,#230291,#230292,#230293,#230294,
#230295,#230296,#230297,#230298,#230299,#230300,#230301,#230302,#230303,
#230304,#230305,#230306,#230307,#230308,#230309,#230310,#230311,#230312,
#230313,#230314,#230315,#230316,#230317,#230318,#230319,#230320,#230321,
#230322,#230323,#230324,#230325,#230326,#230327,#230328,#230329,#230330,
#230331,#230332),.UNSPECIFIED.,.F.,.F.,(4,3,3,3,3,3,3,3,3,3,3,3,3,3,3,3,
3,4),(0.,4.30706237876165E-5,8.47417087707063E-5,0.000124159989206986,0.000160467076291406,
0.000170998382116689,0.000182414994733778,0.000213747977645862,0.000242415955902294,
0.000256497573175035,0.000259169422895608,0.000261757777312413,0.000289965130403309,
0.000301877270772897,0.000321937017503139,0.000326951954185699,0.00033447435920954,
0.000341996764233381),.UNSPECIFIED.);
#5008=B_SPLINE_CURVE_WITH_KNOTS('',3,(#230333,#230334,#230335,#230336,#230337,
#230338,#230339,#230340,#230341,#230342,#230343,#230344,#230345,#230346,
#230347,#230348,#230349,#230350,#230351,#230352,#230353,#230354,#230355,
#230356,#230357,#230358,#230359,#230360,#230361,#230362,#230363,#230364,
#230365,#230366,#230367,#230368,#230369,#230370,#230371,#230372,#230373,
#230374,#230375,#230376,#230377,#230378,#230379,#230380,#230381,#230382,
#230383,#230384),.UNSPECIFIED.,.F.,.F.,(4,3,3,3,3,3,3,3,3,3,3,3,3,3,3,3,
3,4),(0.,2.58457451683339E-5,4.25394446195427E-5,6.46659869686937E-5,7.57292581432692E-5,
8.12608937305569E-5,8.26438026273789E-5,8.67925293178447E-5,0.000116015624427496,
0.000130188793976767,0.000151886926306228,0.000161963651211283,0.000162735992470959,
0.000173585058635689,0.000212487880461562,0.000255238173512928,0.000301397761149189,
0.000347170117271379),.UNSPECIFIED.);
#5009=B_SPLINE_CURVE_WITH_KNOTS('',3,(#230386,#230387,#230388,#230389,#230390,
#230391,#230392,#230393,#230394,#230395,#230396,#230397,#230398,#230399,
#230400,#230401,#230402,#230403,#230404,#230405,#230406,#230407,#230408,
#230409,#230410,#230411,#230412,#230413,#230414,#230415,#230416,#230417,
#230418,#230419,#230420,#230421,#230422,#230423,#230424,#230425,#230426,
#230427,#230428,#230429,#230430,#230431),.UNSPECIFIED.,.F.,.F.,(4,3,3,3,
3,3,3,3,3,3,3,3,3,3,3,4),(0.,2.57218161995344E-5,4.21568322568466E-5,6.45873314617301E-5,
7.58025810641718E-5,8.14102058653927E-5,8.28121120656979E-5,8.70178306666136E-5,
0.000116081955657677,0.00013052674599992,0.000162394111022036,0.000174035661333227,
0.000213138396957751,0.000256116935432942,0.000302406662855227,0.000348071322666453),
 .UNSPECIFIED.);
#5010=B_SPLINE_CURVE_WITH_KNOTS('',3,(#230432,#230433,#230434,#230435,#230436,
#230437,#230438,#230439,#230440,#230441,#230442,#230443,#230444,#230445,
#230446,#230447,#230448,#230449,#230450,#230451,#230452,#230453,#230454,
#230455,#230456,#230457,#230458,#230459,#230460,#230461,#230462,#230463,
#230464,#230465,#230466,#230467,#230468,#230469,#230470,#230471,#230472,
#230473,#230474,#230475,#230476,#230477,#230478,#230479,#230480,#230481,
#230482,#230483),.UNSPECIFIED.,.F.,.F.,(4,3,3,3,3,3,3,3,3,3,3,3,3,3,3,3,
3,4),(0.,4.29652152186797E-5,8.44519107576635E-5,0.000123669830870363,0.000159788877364213,
0.000170558847912623,0.000181218775907163,0.000181960046452394,0.00021446006264392,
0.000244755726199048,0.000255838271868943,0.000258503253867578,0.000261084955178756,
0.000289370476647024,0.00030110132550201,0.000321109510663637,0.00033111360324445,
0.000341117695825264),.UNSPECIFIED.);
#5011=B_SPLINE_CURVE_WITH_KNOTS('',3,(#230485,#230486,#230487,#230488,#230489,
#230490,#230491,#230492,#230493,#230494,#230495,#230496,#230497,#230498,
#230499,#230500,#230501,#230502,#230503,#230504,#230505,#230506,#230507,
#230508,#230509,#230510,#230511,#230512,#230513,#230514,#230515,#230516,
#230517,#230518,#230519,#230520,#230521,#230522,#230523,#230524,#230525,
#230526,#230527,#230528,#230529,#230530,#230531,#230532,#230533,#230534,
#230535,#230536),.UNSPECIFIED.,.F.,.F.,(4,3,3,3,3,3,3,3,3,3,3,3,3,3,3,3,
3,4),(8.67361737988404E-19,4.30706237860763E-5,8.47417087680201E-5,0.000124159989203277,
0.000160467076286602,0.00017099838211669,0.000182414994733777,0.000213747977645865,
0.00024241595590321,0.00025649757317504,0.000259169422895614,0.000261757777312419,
0.000289965130402967,0.000301877270772905,0.000321937017503148,0.000326951954185708,
0.000334474359209549,0.00034199676423339),.UNSPECIFIED.);
#5012=B_SPLINE_CURVE_WITH_KNOTS('',3,(#230537,#230538,#230539,#230540,#230541,
#230542,#230543,#230544,#230545,#230546,#230547,#230548,#230549,#230550,
#230551,#230552,#230553,#230554,#230555,#230556,#230557,#230558,#230559,
#230560,#230561,#230562,#230563,#230564,#230565,#230566,#230567,#230568,
#230569,#230570,#230571,#230572,#230573,#230574,#230575,#230576,#230577,
#230578,#230579,#230580,#230581,#230582,#230583,#230584,#230585,#230586,
#230587,#230588),.UNSPECIFIED.,.F.,.F.,(4,3,3,3,3,3,3,3,3,3,3,3,3,3,3,3,
3,4),(6.93889390390723E-18,2.58457451701831E-5,4.25394446195401E-5,6.46659869686908E-5,
7.57292581432661E-5,8.12608937305538E-5,8.26438026273757E-5,8.67925293178415E-5,
0.000116015624427578,0.000130188793976759,0.000151886926306217,0.000161963651211268,
0.000162735992470947,0.000173585058635676,0.000212487880458399,0.000255238173505916,
0.000301397761136468,0.000347170117271362),.UNSPECIFIED.);
#5013=B_SPLINE_CURVE_WITH_KNOTS('',3,(#230590,#230591,#230592,#230593,#230594,
#230595,#230596,#230597,#230598,#230599,#230600,#230601,#230602,#230603,
#230604,#230605,#230606,#230607,#230608,#230609,#230610,#230611,#230612,
#230613,#230614,#230615,#230616,#230617,#230618,#230619,#230620,#230621,
#230622,#230623,#230624,#230625,#230626,#230627,#230628,#230629,#230630,
#230631,#230632,#230633,#230634,#230635),.UNSPECIFIED.,.F.,.F.,(4,3,3,3,
3,3,3,3,3,3,3,3,3,3,3,4),(6.93889390390723E-18,2.57218161998122E-5,4.21568322568062E-5,
6.45873314617115E-5,7.58025810641641E-5,8.14102058653904E-5,8.2812112065697E-5,
8.70178306666167E-5,0.000116081955658388,0.000130526745999922,0.000162394111022033,
0.000174035661333226,0.000213138396956944,0.000256116935431236,0.000302406662852219,
0.000348071322666445),.UNSPECIFIED.);
#5014=B_SPLINE_CURVE_WITH_KNOTS('',3,(#230636,#230637,#230638,#230639,#230640,
#230641,#230642,#230643,#230644,#230645,#230646,#230647,#230648,#230649,
#230650,#230651,#230652,#230653,#230654,#230655,#230656,#230657,#230658,
#230659,#230660,#230661,#230662,#230663,#230664,#230665,#230666,#230667,
#230668,#230669,#230670,#230671,#230672,#230673,#230674,#230675,#230676,
#230677,#230678,#230679,#230680,#230681,#230682,#230683,#230684,#230685,
#230686,#230687),.UNSPECIFIED.,.F.,.F.,(4,3,3,3,3,3,3,3,3,3,3,3,3,3,3,3,
3,4),(0.,4.29652152192065E-5,8.44519107585664E-5,0.000123669830871595,0.000159788877365913,
0.000170558847912624,0.000181218775907164,0.000181960046452394,0.000214460062644216,
0.000244755726200167,0.000255838271868943,0.000258503253867578,0.000261084955178756,
0.000289370476646725,0.000301101325502009,0.000321109510663636,0.000331113603244449,
0.000341117695825263),.UNSPECIFIED.);
#5015=B_SPLINE_CURVE_WITH_KNOTS('',3,(#230689,#230690,#230691,#230692,#230693,
#230694,#230695,#230696,#230697,#230698,#230699,#230700,#230701,#230702,
#230703,#230704,#230705,#230706,#230707,#230708,#230709,#230710,#230711,
#230712,#230713,#230714,#230715,#230716,#230717,#230718,#230719,#230720,
#230721,#230722,#230723,#230724,#230725,#230726,#230727,#230728,#230729,
#230730,#230731,#230732,#230733,#230734,#230735,#230736,#230737,#230738,
#230739,#230740),.UNSPECIFIED.,.F.,.F.,(4,3,3,3,3,3,3,3,3,3,3,3,3,3,3,3,
3,4),(0.,4.30706237839992E-5,8.47417087643213E-5,0.000124159989198158,0.000160467076279949,
0.000170998382116701,0.00018241499473378,0.000213747977645876,0.000242415955902872,
0.000256497573175051,0.000259169422895625,0.00026175777731243,0.000289965130403972,
0.000301877270772916,0.000321937017503159,0.00032695195418572,0.000334474359209561,
0.000341996764233402),.UNSPECIFIED.);
#5016=B_SPLINE_CURVE_WITH_KNOTS('',3,(#230741,#230742,#230743,#230744,#230745,
#230746,#230747,#230748,#230749,#230750,#230751,#230752,#230753,#230754,
#230755,#230756,#230757,#230758,#230759,#230760,#230761,#230762,#230763,
#230764,#230765,#230766,#230767,#230768,#230769,#230770,#230771,#230772,
#230773,#230774,#230775,#230776,#230777,#230778,#230779,#230780,#230781,
#230782,#230783,#230784,#230785,#230786,#230787,#230788,#230789,#230790,
#230791,#230792),.UNSPECIFIED.,.F.,.F.,(4,3,3,3,3,3,3,3,3,3,3,3,3,3,3,3,
3,4),(3.46944695195361E-18,2.58457451697252E-5,4.25394446195546E-5,6.46659869687025E-5,
7.57292581432765E-5,8.12608937305634E-5,8.26438026273852E-5,8.67925293178504E-5,
0.000116015624427319,0.000130188793976774,0.000151886926306236,0.000161963651211266,
0.000162735992470966,0.000173585058635697,0.000212487880459449,0.0002552381735094,
0.000301397761145159,0.000347170117271374),.UNSPECIFIED.);
#5017=B_SPLINE_CURVE_WITH_KNOTS('',3,(#230794,#230795,#230796,#230797,#230798,
#230799,#230800,#230801,#230802,#230803,#230804,#230805,#230806,#230807,
#230808,#230809,#230810,#230811,#230812,#230813,#230814,#230815,#230816,
#230817,#230818,#230819,#230820,#230821,#230822,#230823,#230824,#230825,
#230826,#230827,#230828,#230829,#230830,#230831,#230832,#230833,#230834,
#230835,#230836,#230837,#230838,#230839),.UNSPECIFIED.,.F.,.F.,(4,3,3,3,
3,3,3,3,3,3,3,3,3,3,3,4),(0.,2.57218161988346E-5,4.21568322566952E-5,6.45873314616517E-5,
7.580258106413E-5,8.14102058653691E-5,8.28121120656789E-5,8.70178306666082E-5,
0.000116081955657482,0.000130526745999912,0.000162394111022032,0.000174035661333216,
0.000213138396961443,0.000256116935440209,0.000302406662866123,0.000348071322666431),
 .UNSPECIFIED.);
#5018=B_SPLINE_CURVE_WITH_KNOTS('',3,(#230840,#230841,#230842,#230843,#230844,
#230845,#230846,#230847,#230848,#230849,#230850,#230851,#230852,#230853,
#230854,#230855,#230856,#230857,#230858,#230859,#230860,#230861,#230862,
#230863,#230864,#230865,#230866,#230867,#230868,#230869,#230870,#230871,
#230872,#230873,#230874,#230875,#230876,#230877,#230878,#230879,#230880,
#230881,#230882,#230883,#230884,#230885,#230886,#230887,#230888,#230889,
#230890,#230891),.UNSPECIFIED.,.F.,.F.,(4,3,3,3,3,3,3,3,3,3,3,3,3,3,3,3,
3,4),(1.30104260698261E-18,4.29652152148209E-5,8.44519107512452E-5,0.000123669830862091,
0.000159788877354504,0.000170558847912628,0.000181218775907167,0.000181960046452412,
0.000214460062643743,0.000244755726199073,0.00025583827186894,0.000258503253867575,
0.000261084955178753,0.000289370476647586,0.000301101325502003,0.000321109510663628,
0.00033111360324444,0.000341117695825253),.UNSPECIFIED.);
#5019=B_SPLINE_CURVE_WITH_KNOTS('',3,(#230893,#230894,#230895,#230896,#230897,
#230898,#230899,#230900,#230901,#230902,#230903,#230904,#230905,#230906,
#230907,#230908,#230909,#230910,#230911,#230912,#230913,#230914,#230915,
#230916,#230917,#230918,#230919,#230920,#230921,#230922,#230923,#230924,
#230925,#230926,#230927,#230928,#230929,#230930,#230931,#230932,#230933,
#230934,#230935,#230936,#230937,#230938,#230939,#230940,#230941,#230942,
#230943,#230944),.UNSPECIFIED.,.F.,.F.,(4,3,3,3,3,3,3,3,3,3,3,3,3,3,3,3,
3,4),(0.,4.30706237882036E-5,8.47417087719642E-5,0.000124159989209034,0.000160467076294394,
0.000170998382116691,0.00018241499473377,0.000213747977645865,0.000242415955902961,
0.00025649757317504,0.000259169422895613,0.000261757777312419,0.00028996513040394,
0.000301877270772904,0.000321937017503146,0.000326951954185707,0.000334474359209548,
0.000341996764233389),.UNSPECIFIED.);
#5020=B_SPLINE_CURVE_WITH_KNOTS('',3,(#230945,#230946,#230947,#230948,#230949,
#230950,#230951,#230952,#230953,#230954,#230955,#230956,#230957,#230958,
#230959,#230960,#230961,#230962,#230963,#230964,#230965,#230966,#230967,
#230968,#230969,#230970,#230971,#230972,#230973,#230974,#230975,#230976,
#230977,#230978,#230979,#230980,#230981,#230982,#230983,#230984,#230985,
#230986,#230987,#230988,#230989,#230990,#230991,#230992,#230993,#230994,
#230995,#230996),.UNSPECIFIED.,.F.,.F.,(4,3,3,3,3,3,3,3,3,3,3,3,3,3,3,3,
3,4),(3.46944695195361E-18,2.58457451678337E-5,4.25394446195919E-5,6.46659869687144E-5,
7.57292581432757E-5,8.12608937305563E-5,8.26438026273765E-5,8.67925293178369E-5,
0.000116015624427211,0.000130188793976754,0.000151886926306212,0.000161963651211262,
0.000162735992470941,0.00017358505863567,0.00021248788046187,0.000255238173513225,
0.000301397761148772,0.000347170117271356),.UNSPECIFIED.);
#5021=B_SPLINE_CURVE_WITH_KNOTS('',3,(#230998,#230999,#231000,#231001,#231002,
#231003,#231004,#231005,#231006,#231007,#231008,#231009,#231010,#231011,
#231012,#231013,#231014,#231015,#231016,#231017,#231018,#231019,#231020,
#231021,#231022,#231023,#231024,#231025,#231026,#231027,#231028,#231029,
#231030,#231031,#231032,#231033,#231034,#231035,#231036,#231037,#231038,
#231039,#231040,#231041,#231042,#231043),.UNSPECIFIED.,.F.,.F.,(4,3,3,3,
3,3,3,3,3,3,3,3,3,3,3,4),(0.,2.57218162018153E-5,4.21568322567147E-5,6.45873314616719E-5,
7.58025810641505E-5,8.14102058653898E-5,8.28121120656996E-5,8.70178306666291E-5,
0.000116081955659704,0.000130526745999944,0.000162394111022071,0.000174035661333258,
0.000213138396959943,0.0002561169354372,0.000302406662861553,0.000348071322666499),
 .UNSPECIFIED.);
#5022=B_SPLINE_CURVE_WITH_KNOTS('',3,(#231044,#231045,#231046,#231047,#231048,
#231049,#231050,#231051,#231052,#231053,#231054,#231055,#231056,#231057,
#231058,#231059,#231060,#231061,#231062,#231063,#231064,#231065,#231066,
#231067,#231068,#231069,#231070,#231071,#231072,#231073,#231074,#231075,
#231076,#231077,#231078,#231079,#231080,#231081,#231082,#231083,#231084,
#231085,#231086,#231087,#231088,#231089,#231090,#231091,#231092,#231093,
#231094,#231095),.UNSPECIFIED.,.F.,.F.,(4,3,3,3,3,3,3,3,3,3,3,3,3,3,3,3,
3,4),(8.67361737988404E-19,4.2965215210266E-5,8.44519107438952E-5,0.000123669830853,
0.000159788877344359,0.000170558847912642,0.000181218775907182,0.000181960046452411,
0.000214460062643778,0.000244755726198623,0.000255838271868959,0.000258503253867594,
0.000261084955178771,0.000289370476647211,0.000301101325502024,0.00032110951066365,
0.000331113603244463,0.000341117695825276),.UNSPECIFIED.);
#5023=B_SPLINE_CURVE_WITH_KNOTS('',3,(#231097,#231098,#231099,#231100,#231101,
#231102,#231103,#231104,#231105,#231106,#231107,#231108,#231109,#231110,
#231111,#231112,#231113,#231114,#231115,#231116,#231117,#231118,#231119,
#231120,#231121,#231122,#231123,#231124,#231125,#231126,#231127,#231128,
#231129,#231130,#231131,#231132,#231133,#231134,#231135,#231136,#231137,
#231138,#231139,#231140,#231141,#231142,#231143,#231144,#231145,#231146,
#231147,#231148),.UNSPECIFIED.,.F.,.F.,(4,3,3,3,3,3,3,3,3,3,3,3,3,3,3,3,
3,4),(0.,4.30706237851929E-5,8.47417087663985E-5,0.000124159989200908,0.000160467076283494,
0.000170998382116701,0.000182414994733797,0.000213747977645873,0.000242415955903371,
0.000256497573175046,0.00025916942289562,0.000261757777312425,0.000289965130403631,
0.000301877270772908,0.00032193701750315,0.000326951954185711,0.000334474359209551,
0.000341996764233392),.UNSPECIFIED.);
#5024=B_SPLINE_CURVE_WITH_KNOTS('',3,(#231149,#231150,#231151,#231152,#231153,
#231154,#231155,#231156,#231157,#231158,#231159,#231160,#231161,#231162,
#231163,#231164,#231165,#231166,#231167,#231168,#231169,#231170,#231171,
#231172,#231173,#231174,#231175,#231176,#231177,#231178,#231179,#231180,
#231181,#231182,#231183,#231184,#231185,#231186,#231187,#231188,#231189,
#231190,#231191,#231192,#231193,#231194,#231195,#231196,#231197,#231198,
#231199,#231200),.UNSPECIFIED.,.F.,.F.,(4,3,3,3,3,3,3,3,3,3,3,3,3,3,3,3,
3,4),(3.46944695195361E-18,2.58457451697524E-5,4.25394446195375E-5,6.46659869686935E-5,
7.57292581432715E-5,8.12608937305605E-5,8.26438026273827E-5,8.67925293178494E-5,
0.000116015624427668,0.000130188793976772,0.000151886926306234,0.000161963651211282,
0.000162735992470965,0.000173585058635695,0.000212487880458633,0.000255238173507009,
0.000301397761139473,0.000347170117271371),.UNSPECIFIED.);
#5025=B_SPLINE_CURVE_WITH_KNOTS('',3,(#231202,#231203,#231204,#231205,#231206,
#231207,#231208,#231209,#231210,#231211,#231212,#231213,#231214,#231215,
#231216,#231217,#231218,#231219,#231220,#231221,#231222,#231223,#231224,
#231225,#231226,#231227,#231228,#231229,#231230,#231231,#231232,#231233,
#231234,#231235,#231236,#231237,#231238,#231239,#231240,#231241,#231242,
#231243,#231244,#231245,#231246,#231247),.UNSPECIFIED.,.F.,.F.,(4,3,3,3,
3,3,3,3,3,3,3,3,3,3,3,4),(0.,2.57218161998829E-5,4.21568322568464E-5,6.45873314617307E-5,
7.58025810641729E-5,8.14102058653939E-5,8.28121120656992E-5,8.7017830666615E-5,
0.000116081955659212,0.000130526745999922,0.000162394111022053,0.00017403566133323,
0.000213138396958018,0.000256116935433331,0.000302406662855306,0.000348071322666447),
 .UNSPECIFIED.);
#5026=B_SPLINE_CURVE_WITH_KNOTS('',3,(#231248,#231249,#231250,#231251,#231252,
#231253,#231254,#231255,#231256,#231257,#231258,#231259,#231260,#231261,
#231262,#231263,#231264,#231265,#231266,#231267,#231268,#231269,#231270,
#231271,#231272,#231273,#231274,#231275,#231276,#231277,#231278,#231279,
#231280,#231281,#231282,#231283,#231284,#231285,#231286,#231287,#231288,
#231289,#231290,#231291,#231292,#231293,#231294,#231295,#231296,#231297,
#231298,#231299),.UNSPECIFIED.,.F.,.F.,(4,3,3,3,3,3,3,3,3,3,3,3,3,3,3,3,
3,4),(0.,4.29652152128983E-5,8.44519107483271E-5,0.000123669830858996,0.000159788877351773,
0.000170558847912631,0.00018121877590717,0.000181960046452391,0.000214460062644109,
0.000244755726200095,0.000255838271868941,0.000258503253867576,0.000261084955178753,
0.000289370476647502,0.000301101325502003,0.000321109510663627,0.000331113603244439,
0.000341117695825252),.UNSPECIFIED.);
#5027=B_SPLINE_CURVE_WITH_KNOTS('',3,(#231301,#231302,#231303,#231304,#231305,
#231306,#231307,#231308,#231309,#231310,#231311,#231312,#231313,#231314,
#231315,#231316,#231317,#231318,#231319,#231320,#231321,#231322,#231323,
#231324,#231325,#231326,#231327,#231328,#231329,#231330,#231331,#231332,
#231333,#231334,#231335,#231336,#231337,#231338,#231339,#231340,#231341,
#231342,#231343,#231344,#231345,#231346,#231347,#231348,#231349,#231350,
#231351,#231352),.UNSPECIFIED.,.F.,.F.,(4,3,3,3,3,3,3,3,3,3,3,3,3,3,3,3,
3,4),(0.,4.30706237880135E-5,8.4741708771494E-5,0.000124159989208263,0.000160467076293188,
0.000170998382116689,0.000182414994733767,0.000213747977645861,0.000242415955903085,
0.000256497573175034,0.000259169422895607,0.000261757777312412,0.000289965130403409,
0.000301877270772895,0.000321937017503137,0.000326951954185697,0.000334474359209537,
0.000341996764233378),.UNSPECIFIED.);
#5028=B_SPLINE_CURVE_WITH_KNOTS('',3,(#231353,#231354,#231355,#231356,#231357,
#231358,#231359,#231360,#231361,#231362,#231363,#231364,#231365,#231366,
#231367,#231368,#231369,#231370,#231371,#231372,#231373,#231374,#231375,
#231376,#231377,#231378,#231379,#231380,#231381,#231382,#231383,#231384,
#231385,#231386,#231387,#231388,#231389,#231390,#231391,#231392,#231393,
#231394,#231395,#231396,#231397,#231398,#231399,#231400,#231401,#231402,
#231403,#231404),.UNSPECIFIED.,.F.,.F.,(4,3,3,3,3,3,3,3,3,3,3,3,3,3,3,3,
3,4),(0.,2.5845745169089E-5,4.25394446195701E-5,6.46659869687081E-5,7.57292581432771E-5,
8.12608937305616E-5,8.26438026273827E-5,8.6792529317846E-5,0.000116015624427623,
0.000130188793976769,0.000151886926306231,0.00016196365121128,0.000162735992470961,
0.000173585058635692,0.000212487880461807,0.000255238173513942,0.000301397761151968,
0.000347170117271371),.UNSPECIFIED.);
#5029=B_SPLINE_CURVE_WITH_KNOTS('',3,(#231406,#231407,#231408,#231409,#231410,
#231411,#231412,#231413,#231414,#231415,#231416,#231417,#231418,#231419,
#231420,#231421,#231422,#231423,#231424,#231425,#231426,#231427,#231428,
#231429,#231430,#231431,#231432,#231433,#231434,#231435,#231436,#231437,
#231438,#231439,#231440,#231441,#231442,#231443,#231444,#231445,#231446,
#231447,#231448,#231449,#231450,#231451),.UNSPECIFIED.,.F.,.F.,(4,3,3,3,
3,3,3,3,3,3,3,3,3,3,3,4),(0.,2.5721816199856E-5,4.21568322568771E-5,6.45873314617458E-5,
7.58025810641801E-5,8.14102058653973E-5,8.28121120657016E-5,8.70178306666145E-5,
0.000116081955658527,0.000130526745999922,0.000162394111022043,0.000174035661333229,
0.00021313839695968,0.000256116935436711,0.000302406662860802,0.000348071322666442),
 .UNSPECIFIED.);
#5030=B_SPLINE_CURVE_WITH_KNOTS('',3,(#231452,#231453,#231454,#231455,#231456,
#231457,#231458,#231459,#231460,#231461,#231462,#231463,#231464,#231465,
#231466,#231467,#231468,#231469,#231470,#231471,#231472,#231473,#231474,
#231475,#231476,#231477,#231478,#231479,#231480,#231481,#231482,#231483,
#231484,#231485,#231486,#231487,#231488,#231489,#231490,#231491,#231492,
#231493,#231494,#231495,#231496,#231497,#231498,#231499,#231500,#231501,
#231502,#231503),.UNSPECIFIED.,.F.,.F.,(4,3,3,3,3,3,3,3,3,3,3,3,3,3,3,3,
3,4),(4.33680868994202E-19,4.29652152140341E-5,8.44519107501717E-5,0.000123669830861157,
0.000159788877354104,0.000170558847912632,0.000181218775907171,0.000181960046452407,
0.000214460062644171,0.000244755726200186,0.000255838271868944,0.000258503253867579,
0.000261084955178757,0.000289370476646964,0.000301101325502007,0.000321109510663632,
0.000331113603244444,0.000341117695825257),.UNSPECIFIED.);
#5031=B_SPLINE_CURVE_WITH_KNOTS('',3,(#231505,#231506,#231507,#231508,#231509,
#231510,#231511,#231512,#231513,#231514,#231515,#231516,#231517,#231518,
#231519,#231520,#231521,#231522,#231523,#231524,#231525,#231526,#231527,
#231528,#231529,#231530,#231531,#231532,#231533,#231534,#231535,#231536,
#231537,#231538,#231539,#231540,#231541,#231542,#231543,#231544,#231545,
#231546,#231547,#231548,#231549,#231550,#231551,#231552,#231553,#231554,
#231555,#231556),.UNSPECIFIED.,.F.,.F.,(4,3,3,3,3,3,3,3,3,3,3,3,3,3,3,3,
3,4),(0.,4.30706237871702E-5,8.47417087699776E-5,0.000124159989206078,0.000160467076290317,
0.000170998382116687,0.000182414994733769,0.000213747977645862,0.000242415955904907,
0.000256497573175036,0.00025916942289561,0.000261757777312415,0.000289965130402048,
0.000301877270772901,0.000321937017503143,0.000326951954185704,0.000334474359209545,
0.000341996764233386),.UNSPECIFIED.);
#5032=B_SPLINE_CURVE_WITH_KNOTS('',3,(#231557,#231558,#231559,#231560,#231561,
#231562,#231563,#231564,#231565,#231566,#231567,#231568,#231569,#231570,
#231571,#231572,#231573,#231574,#231575,#231576,#231577,#231578,#231579,
#231580,#231581,#231582,#231583,#231584,#231585,#231586,#231587,#231588,
#231589,#231590,#231591,#231592,#231593,#231594,#231595,#231596,#231597,
#231598,#231599,#231600,#231601,#231602,#231603,#231604,#231605,#231606,
#231607,#231608),.UNSPECIFIED.,.F.,.F.,(4,3,3,3,3,3,3,3,3,3,3,3,3,3,3,3,
3,4),(0.,2.58457451693448E-5,4.25394446196001E-5,6.46659869687223E-5,7.57292581432835E-5,
8.1260893730564E-5,8.26438026273842E-5,8.67925293178446E-5,0.000116015624427668,
0.000130188793976767,0.000151886926306228,0.000161963651211283,0.000162735992470959,
0.000173585058635689,0.00021248788045699,0.00025523817350245,0.000301397761129275,
0.000347170117271378),.UNSPECIFIED.);
#5033=B_SPLINE_CURVE_WITH_KNOTS('',3,(#231610,#231611,#231612,#231613,#231614,
#231615,#231616,#231617,#231618,#231619,#231620,#231621,#231622,#231623,
#231624,#231625,#231626,#231627,#231628,#231629,#231630,#231631,#231632,
#231633,#231634,#231635,#231636,#231637,#231638,#231639,#231640,#231641,
#231642,#231643,#231644,#231645,#231646,#231647,#231648,#231649,#231650,
#231651,#231652,#231653,#231654,#231655),.UNSPECIFIED.,.F.,.F.,(4,3,3,3,
3,3,3,3,3,3,3,3,3,3,3,4),(8.67361737988404E-19,2.57218162006469E-5,4.21568322567888E-5,
6.45873314617057E-5,7.58025810641642E-5,8.14102058653934E-5,8.28121120657007E-5,
8.70178306666226E-5,0.000116081955659052,0.000130526745999934,0.000162394111022055,
0.000174035661333244,0.000213138396957381,0.000256116935431866,0.000302406662852459,
0.000348071322666488),.UNSPECIFIED.);
#5034=B_SPLINE_CURVE_WITH_KNOTS('',3,(#231656,#231657,#231658,#231659,#231660,
#231661,#231662,#231663,#231664,#231665,#231666,#231667,#231668,#231669,
#231670,#231671,#231672,#231673,#231674,#231675,#231676,#231677,#231678,
#231679,#231680,#231681,#231682,#231683,#231684,#231685,#231686,#231687,
#231688,#231689,#231690,#231691,#231692,#231693,#231694,#231695,#231696,
#231697,#231698,#231699,#231700,#231701,#231702,#231703,#231704,#231705,
#231706,#231707),.UNSPECIFIED.,.F.,.F.,(4,3,3,3,3,3,3,3,3,3,3,3,3,3,3,3,
3,4),(0.,4.2965215222015E-5,8.44519107628343E-5,0.000123669830876255,0.000159788877370164,
0.000170558847912636,0.000181218775907176,0.000181960046452415,0.000214460062643924,
0.00024475572619964,0.000255838271868954,0.000258503253867589,0.000261084955178766,
0.000289370476647491,0.000301101325502019,0.000321109510663645,0.000331113603244458,
0.000341117695825272),.UNSPECIFIED.);
#5035=B_SPLINE_CURVE_WITH_KNOTS('',3,(#231709,#231710,#231711,#231712,#231713,
#231714,#231715,#231716,#231717,#231718,#231719,#231720,#231721,#231722,
#231723,#231724,#231725,#231726,#231727,#231728,#231729,#231730,#231731,
#231732,#231733,#231734,#231735,#231736,#231737,#231738,#231739,#231740,
#231741,#231742,#231743,#231744,#231745,#231746,#231747,#231748,#231749,
#231750,#231751,#231752,#231753,#231754,#231755,#231756,#231757,#231758,
#231759,#231760),.UNSPECIFIED.,.F.,.F.,(4,3,3,3,3,3,3,3,3,3,3,3,3,3,3,3,
3,4),(3.09377807083354E-18,4.30706237851843E-5,8.47417087666321E-5,0.000124159989201714,
0.00016046707628494,0.00017099838211668,0.000182414994733754,0.000213747977645856,
0.000242415955903085,0.000256497573175032,0.000259169422895605,0.000261757777312411,
0.000289965130403707,0.000301877270772897,0.000321937017503141,0.000326951954185701,
0.000334474359209543,0.000341996764233384),.UNSPECIFIED.);
#5036=B_SPLINE_CURVE_WITH_KNOTS('',3,(#231761,#231762,#231763,#231764,#231765,
#231766,#231767,#231768,#231769,#231770,#231771,#231772,#231773,#231774,
#231775,#231776,#231777,#231778,#231779,#231780,#231781,#231782,#231783,
#231784,#231785,#231786,#231787,#231788,#231789,#231790,#231791,#231792,
#231793,#231794,#231795,#231796,#231797,#231798,#231799,#231800,#231801,
#231802,#231803,#231804,#231805,#231806,#231807,#231808,#231809,#231810,
#231811,#231812),.UNSPECIFIED.,.F.,.F.,(4,3,3,3,3,3,3,3,3,3,3,3,3,3,3,3,
3,4),(2.76132740804902E-19,2.58457451684212E-5,4.25394446196281E-5,6.4665986968732E-5,
7.5729258143284E-5,8.126089373056E-5,8.2643802627379E-5,8.6792529317836E-5,
0.000116015624427268,0.000130188793976754,0.000151886926306213,0.000161963651211274,
0.000162735992470942,0.000173585058635672,0.000212487880460351,0.00025523817351116,
0.000301397761147902,0.000347170117271357),.UNSPECIFIED.);
#5037=B_SPLINE_CURVE_WITH_KNOTS('',3,(#231814,#231815,#231816,#231817,#231818,
#231819,#231820,#231821,#231822,#231823,#231824,#231825,#231826,#231827,
#231828,#231829,#231830,#231831,#231832,#231833,#231834,#231835,#231836,
#231837,#231838,#231839,#231840,#231841,#231842,#231843,#231844,#231845,
#231846,#231847,#231848,#231849,#231850,#231851,#231852,#231853,#231854,
#231855,#231856,#231857,#231858,#231859),.UNSPECIFIED.,.F.,.F.,(4,3,3,3,
3,3,3,3,3,3,3,3,3,3,3,4),(2.74438674910393E-19,2.57218161985759E-5,4.215683225698E-5,
6.45873314618026E-5,7.58025810642139E-5,8.14102058654196E-5,8.2812112065721E-5,
8.70178306666252E-5,0.000116081955658136,0.000130526745999938,0.000162394111022044,
0.00017403566133325,0.000213138396957668,0.000256116935432663,0.000302406662854469,
0.000348071322666499),.UNSPECIFIED.);
#5038=B_SPLINE_CURVE_WITH_KNOTS('',3,(#231860,#231861,#231862,#231863,#231864,
#231865,#231866,#231867,#231868,#231869,#231870,#231871,#231872,#231873,
#231874,#231875,#231876,#231877,#231878,#231879,#231880,#231881,#231882,
#231883,#231884,#231885,#231886,#231887,#231888,#231889,#231890,#231891,
#231892,#231893,#231894,#231895,#231896,#231897,#231898,#231899,#231900,
#231901,#231902,#231903,#231904,#231905,#231906,#231907,#231908,#231909,
#231910,#231911),.UNSPECIFIED.,.F.,.F.,(4,3,3,3,3,3,3,3,3,3,3,3,3,3,3,3,
3,4),(0.,4.29652152154259E-5,8.44519107524018E-5,0.000123669830863876,0.000159788877357041,
0.000170558847912633,0.000181218775907173,0.000181960046452409,0.000214460062643776,
0.000244755726199061,0.00025583827186895,0.000258503253867585,0.000261084955178762,
0.000289370476647126,0.000301101325502014,0.00032110951066364,0.000331113603244453,
0.000341117695825266),.UNSPECIFIED.);
#5039=B_SPLINE_CURVE_WITH_KNOTS('',3,(#231913,#231914,#231915,#231916,#231917,
#231918,#231919,#231920,#231921,#231922,#231923,#231924,#231925,#231926,
#231927,#231928,#231929,#231930,#231931,#231932,#231933,#231934,#231935,
#231936,#231937,#231938,#231939,#231940,#231941,#231942,#231943,#231944,
#231945,#231946,#231947,#231948,#231949,#231950,#231951,#231952,#231953,
#231954,#231955,#231956,#231957,#231958,#231959,#231960,#231961,#231962,
#231963,#231964),.UNSPECIFIED.,.F.,.F.,(4,3,3,3,3,3,3,3,3,3,3,3,3,3,3,3,
3,4),(4.33680868994202E-19,4.30706237868497E-5,8.47417087694449E-5,0.000124159989205399,
0.000160467076289471,0.000170998382116693,0.000182414994733784,0.000213747977645867,
0.000242415955901955,0.00025649757317504,0.000259169422895613,0.000261757777312419,
0.000289965130404522,0.000301877270772902,0.000321937017503144,0.000326951954185705,
0.000334474359209546,0.000341996764233386),.UNSPECIFIED.);
#5040=B_SPLINE_CURVE_WITH_KNOTS('',3,(#231965,#231966,#231967,#231968,#231969,
#231970,#231971,#231972,#231973,#231974,#231975,#231976,#231977,#231978,
#231979,#231980,#231981,#231982,#231983,#231984,#231985,#231986,#231987,
#231988,#231989,#231990,#231991,#231992,#231993,#231994,#231995,#231996,
#231997,#231998,#231999,#232000,#232001,#232002,#232003,#232004,#232005,
#232006,#232007,#232008,#232009,#232010,#232011,#232012,#232013,#232014,
#232015,#232016),.UNSPECIFIED.,.F.,.F.,(4,3,3,3,3,3,3,3,3,3,3,3,3,3,3,3,
3,4),(0.,2.58457451692491E-5,4.25394446195899E-5,6.46659869687183E-5,7.57292581432825E-5,
8.12608937305646E-5,8.26438026273851E-5,8.67925293178467E-5,0.000116015624427845,
0.00013018879397677,0.000151886926306232,0.000161963651211282,0.000162735992470962,
0.000173585058635693,0.000212487880462679,0.000255238173514224,0.000301397761148888,
0.000347170117271385),.UNSPECIFIED.);
#5041=B_SPLINE_CURVE_WITH_KNOTS('',3,(#232018,#232019,#232020,#232021,#232022,
#232023,#232024,#232025,#232026,#232027,#232028,#232029,#232030,#232031,
#232032,#232033,#232034,#232035,#232036,#232037,#232038,#232039,#232040,
#232041,#232042,#232043,#232044,#232045,#232046,#232047,#232048,#232049,
#232050,#232051,#232052,#232053,#232054,#232055,#232056,#232057,#232058,
#232059,#232060,#232061,#232062,#232063),.UNSPECIFIED.,.F.,.F.,(4,3,3,3,
3,3,3,3,3,3,3,3,3,3,3,4),(0.,2.57218161988135E-5,4.21568322567256E-5,6.45873314616746E-5,
7.58025810641491E-5,8.14102058653863E-5,8.28121120656956E-5,8.70178306666236E-5,
0.000116081955657963,0.000130526745999932,0.000162394111022053,0.00017403566133324,
0.000213138396959429,0.00025611693543614,0.000302406662859657,0.000348071322666484),
 .UNSPECIFIED.);
#5042=B_SPLINE_CURVE_WITH_KNOTS('',3,(#232064,#232065,#232066,#232067,#232068,
#232069,#232070,#232071,#232072,#232073,#232074,#232075,#232076,#232077,
#232078,#232079,#232080,#232081,#232082,#232083,#232084,#232085,#232086,
#232087,#232088,#232089,#232090,#232091,#232092,#232093,#232094,#232095,
#232096,#232097,#232098,#232099,#232100,#232101,#232102,#232103,#232104,
#232105,#232106,#232107,#232108,#232109,#232110,#232111,#232112,#232113,
#232114,#232115),.UNSPECIFIED.,.F.,.F.,(4,3,3,3,3,3,3,3,3,3,3,3,3,3,3,3,
3,4),(0.,4.29652152159573E-5,8.44519107531576E-5,0.000123669830864513,0.000159788877357335,
0.000170558847912642,0.000181218775907181,0.000181960046452405,0.000214460062643898,
0.000244755726199067,0.000255838271868955,0.00025850325386759,0.000261084955178767,
0.000289370476647809,0.000301101325502018,0.000321109510663643,0.000331113603244455,
0.000341117695825268),.UNSPECIFIED.);
#5043=B_SPLINE_CURVE_WITH_KNOTS('',3,(#232117,#232118,#232119,#232120,#232121,
#232122,#232123,#232124,#232125,#232126,#232127,#232128,#232129,#232130,
#232131,#232132,#232133,#232134,#232135,#232136,#232137,#232138,#232139,
#232140,#232141,#232142,#232143,#232144,#232145,#232146,#232147,#232148,
#232149,#232150,#232151,#232152,#232153,#232154,#232155,#232156,#232157,
#232158,#232159,#232160,#232161,#232162,#232163,#232164,#232165,#232166,
#232167,#232168),.UNSPECIFIED.,.F.,.F.,(4,3,3,3,3,3,3,3,3,3,3,3,3,3,3,3,
3,4),(0.,4.30706237860396E-5,8.47417087679563E-5,0.0001241599892032,0.000160467076286543,
0.000170998382116691,0.000182414994733795,0.000213747977645864,0.000242415955901919,
0.000256497573175036,0.00025916942289561,0.000261757777312415,0.000289965130403713,
0.000301877270772899,0.00032193701750314,0.000326951954185701,0.000334474359209541,
0.000341996764233382),.UNSPECIFIED.);
#5044=B_SPLINE_CURVE_WITH_KNOTS('',3,(#232169,#232170,#232171,#232172,#232173,
#232174,#232175,#232176,#232177,#232178,#232179,#232180,#232181,#232182,
#232183,#232184,#232185,#232186,#232187,#232188,#232189,#232190,#232191,
#232192,#232193,#232194,#232195,#232196,#232197,#232198,#232199,#232200,
#232201,#232202,#232203,#232204,#232205,#232206,#232207,#232208,#232209,
#232210,#232211,#232212,#232213,#232214,#232215,#232216,#232217,#232218,
#232219,#232220),.UNSPECIFIED.,.F.,.F.,(4,3,3,3,3,3,3,3,3,3,3,3,3,3,3,3,
3,4),(0.,2.58457451683671E-5,4.25394446195126E-5,6.46659869686776E-5,7.57292581432601E-5,
8.12608937305513E-5,8.26438026273742E-5,8.67925293178426E-5,0.000116015624427412,
0.000130188793976764,0.000151886926306224,0.000161963651211278,0.000162735992470955,
0.000173585058635685,0.000212487880460796,0.000255238173511836,0.000301397761148485,
0.000347170117271367),.UNSPECIFIED.);
#5045=B_SPLINE_CURVE_WITH_KNOTS('',3,(#232222,#232223,#232224,#232225,#232226,
#232227,#232228,#232229,#232230,#232231,#232232,#232233,#232234,#232235,
#232236,#232237,#232238,#232239,#232240,#232241,#232242,#232243,#232244,
#232245,#232246,#232247,#232248,#232249,#232250,#232251,#232252,#232253,
#232254,#232255,#232256,#232257,#232258,#232259,#232260,#232261,#232262,
#232263,#232264,#232265,#232266,#232267),.UNSPECIFIED.,.F.,.F.,(4,3,3,3,
3,3,3,3,3,3,3,3,3,3,3,4),(0.,2.57218162000375E-5,4.21568322568943E-5,6.45873314617579E-5,
7.58025810641896E-5,8.14102058654055E-5,8.28121120657095E-5,8.70178306666214E-5,
0.000116081955658435,0.000130526745999932,0.00016239411102205,0.000174035661333243,
0.000213138396958206,0.000256116935433626,0.000302406662855561,0.000348071322666497),
 .UNSPECIFIED.);
#5046=B_SPLINE_CURVE_WITH_KNOTS('',3,(#232268,#232269,#232270,#232271,#232272,
#232273,#232274,#232275,#232276,#232277,#232278,#232279,#232280,#232281,
#232282,#232283,#232284,#232285,#232286,#232287,#232288,#232289,#232290,
#232291,#232292,#232293,#232294,#232295,#232296,#232297,#232298,#232299,
#232300,#232301,#232302,#232303,#232304,#232305,#232306,#232307,#232308,
#232309,#232310,#232311,#232312,#232313,#232314,#232315,#232316,#232317,
#232318,#232319),.UNSPECIFIED.,.F.,.F.,(4,3,3,3,3,3,3,3,3,3,3,3,3,3,3,3,
3,4),(0.,4.29652152202979E-5,8.44519107602457E-5,0.000123669830873534,0.000159788877367743,
0.000170558847912636,0.000181218775907176,0.000181960046452409,0.000214460062644036,
0.000244755726199992,0.000255838271868954,0.000258503253867589,0.000261084955178767,
0.000289370476647365,0.000301101325502019,0.000321109510663646,0.000331113603244459,
0.000341117695825272),.UNSPECIFIED.);
#5047=B_SPLINE_CURVE_WITH_KNOTS('',3,(#232321,#232322,#232323,#232324,#232325,
#232326,#232327,#232328,#232329,#232330,#232331,#232332,#232333,#232334,
#232335,#232336,#232337,#232338,#232339,#232340,#232341,#232342,#232343,
#232344,#232345,#232346,#232347,#232348,#232349,#232350,#232351,#232352,
#232353,#232354,#232355,#232356,#232357,#232358,#232359,#232360,#232361,
#232362,#232363,#232364,#232365,#232366,#232367,#232368,#232369,#232370,
#232371,#232372),.UNSPECIFIED.,.F.,.F.,(4,3,3,3,3,3,3,3,3,3,3,3,3,3,3,3,
3,4),(3.03576608295941E-18,4.30706237861208E-5,8.47417087680312E-5,0.000124159989203224,
0.000160467076286393,0.000170998382116691,0.000182414994733784,0.000213747977645867,
0.000242415955902087,0.000256497573175044,0.000259169422895617,0.000261757777312423,
0.000289965130404165,0.00030187727077291,0.000321937017503154,0.000326951954185715,
0.000334474359209556,0.000341996764233397),.UNSPECIFIED.);
#5048=B_SPLINE_CURVE_WITH_KNOTS('',3,(#232373,#232374,#232375,#232376,#232377,
#232378,#232379,#232380,#232381,#232382,#232383,#232384,#232385,#232386,
#232387,#232388,#232389,#232390,#232391,#232392,#232393,#232394,#232395,
#232396,#232397,#232398,#232399,#232400,#232401,#232402,#232403,#232404,
#232405,#232406,#232407,#232408,#232409,#232410,#232411,#232412,#232413,
#232414,#232415,#232416,#232417,#232418,#232419,#232420,#232421,#232422,
#232423,#232424),.UNSPECIFIED.,.F.,.F.,(4,3,3,3,3,3,3,3,3,3,3,3,3,3,3,3,
3,4),(0.,2.58457451680044E-5,4.25394446195641E-5,6.46659869687053E-5,7.5729258143276E-5,
8.12608937305613E-5,8.26438026273826E-5,8.67925293178466E-5,0.000116015624427261,
0.00013018879397677,0.000151886926306231,0.000161963651211282,0.000162735992470962,
0.000173585058635693,0.000212487880461109,0.000255238173510755,0.000301397761142687,
0.000347170117271378),.UNSPECIFIED.);
#5049=B_SPLINE_CURVE_WITH_KNOTS('',3,(#232426,#232427,#232428,#232429,#232430,
#232431,#232432,#232433,#232434,#232435,#232436,#232437,#232438,#232439,
#232440,#232441,#232442,#232443,#232444,#232445,#232446,#232447,#232448,
#232449,#232450,#232451,#232452,#232453,#232454,#232455,#232456,#232457,
#232458,#232459,#232460,#232461,#232462,#232463,#232464,#232465,#232466,
#232467,#232468,#232469,#232470,#232471),.UNSPECIFIED.,.F.,.F.,(4,3,3,3,
3,3,3,3,3,3,3,3,3,3,3,4),(0.,2.57218161993042E-5,4.21568322568458E-5,6.45873314617294E-5,
7.58025810641711E-5,8.1410205865392E-5,8.28121120656972E-5,8.70178306666129E-5,
0.000116081955657926,0.000130526745999919,0.000162394111022046,0.000174035661333226,
0.000213138396960043,0.000256116935437413,0.000302406662861798,0.000348071322666454),
 .UNSPECIFIED.);
#5050=B_SPLINE_CURVE_WITH_KNOTS('',3,(#232472,#232473,#232474,#232475,#232476,
#232477,#232478,#232479,#232480,#232481,#232482,#232483,#232484,#232485,
#232486,#232487,#232488,#232489,#232490,#232491,#232492,#232493,#232494,
#232495,#232496,#232497,#232498,#232499,#232500,#232501,#232502,#232503,
#232504,#232505,#232506,#232507,#232508,#232509,#232510,#232511,#232512,
#232513,#232514,#232515,#232516,#232517,#232518,#232519,#232520,#232521,
#232522,#232523),.UNSPECIFIED.,.F.,.F.,(4,3,3,3,3,3,3,3,3,3,3,3,3,3,3,3,
3,4),(4.33680868994202E-19,4.29652152180482E-5,8.44519107565262E-5,0.000123669830868743,
0.000159788877362074,0.000170558847912614,0.000181218775907154,0.000181960046452388,
0.00021446006264368,0.000244755726198699,0.000255838271868931,0.000258503253867566,
0.000261084955178743,0.000289370476647433,0.000301101325501995,0.000321109510663621,
0.000331113603244434,0.000341117695825247),.UNSPECIFIED.);
#5051=B_SPLINE_CURVE_WITH_KNOTS('',3,(#232525,#232526,#232527,#232528,#232529,
#232530,#232531,#232532,#232533,#232534,#232535,#232536,#232537,#232538,
#232539,#232540,#232541,#232542,#232543,#232544,#232545,#232546,#232547,
#232548,#232549,#232550,#232551,#232552,#232553,#232554,#232555,#232556,
#232557,#232558,#232559,#232560,#232561,#232562,#232563,#232564,#232565,
#232566,#232567,#232568,#232569,#232570,#232571,#232572,#232573,#232574,
#232575,#232576),.UNSPECIFIED.,.F.,.F.,(4,3,3,3,3,3,3,3,3,3,3,3,3,3,3,3,
3,4),(0.,4.30706237873825E-5,8.47417087705214E-5,0.000124159989207137,0.000160467076292,
0.000170998382116685,0.000182414994733762,0.000213747977645859,0.000242415955902243,
0.000256497573175034,0.000259169422895608,0.000261757777312413,0.000289965130403732,
0.000301877270772898,0.000321937017503141,0.000326951954185702,0.000334474359209543,
0.000341996764233384),.UNSPECIFIED.);
#5052=B_SPLINE_CURVE_WITH_KNOTS('',3,(#232577,#232578,#232579,#232580,#232581,
#232582,#232583,#232584,#232585,#232586,#232587,#232588,#232589,#232590,
#232591,#232592,#232593,#232594,#232595,#232596,#232597,#232598,#232599,
#232600,#232601,#232602,#232603,#232604,#232605,#232606,#232607,#232608,
#232609,#232610,#232611,#232612,#232613,#232614,#232615,#232616,#232617,
#232618,#232619,#232620,#232621,#232622,#232623,#232624,#232625,#232626,
#232627,#232628),.UNSPECIFIED.,.F.,.F.,(4,3,3,3,3,3,3,3,3,3,3,3,3,3,3,3,
3,4),(3.46944695195361E-18,2.5845745168417E-5,4.25394446196045E-5,6.46659869687246E-5,
7.57292581432846E-5,8.12608937305647E-5,8.26438026273847E-5,8.67925293178447E-5,
0.000116015624427804,0.000130188793976765,0.000151886926306226,0.000161963651211278,
0.000162735992470956,0.000173585058635686,0.0002124878804612,0.000255238173511817,
0.000301397761146479,0.000347170117271368),.UNSPECIFIED.);
#5053=B_SPLINE_CURVE_WITH_KNOTS('',3,(#232630,#232631,#232632,#232633,#232634,
#232635,#232636,#232637,#232638,#232639,#232640,#232641,#232642,#232643,
#232644,#232645,#232646,#232647,#232648,#232649,#232650,#232651,#232652,
#232653,#232654,#232655,#232656,#232657,#232658,#232659,#232660,#232661,
#232662,#232663,#232664,#232665,#232666,#232667,#232668,#232669,#232670,
#232671,#232672,#232673,#232674,#232675),.UNSPECIFIED.,.F.,.F.,(4,3,3,3,
3,3,3,3,3,3,3,3,3,3,3,4),(3.46944695195361E-18,2.57218162005469E-5,4.21568322568319E-5,
6.45873314617224E-5,7.58025810641676E-5,8.14102058653903E-5,8.28121120656959E-5,
8.70178306666129E-5,0.000116081955659199,0.000130526745999918,0.000162394111022043,
0.000174035661333222,0.000213138396958457,0.000256116935434178,0.000302406662856551,
0.000348071322666449),.UNSPECIFIED.);
#5054=B_SPLINE_CURVE_WITH_KNOTS('',3,(#232676,#232677,#232678,#232679,#232680,
#232681,#232682,#232683,#232684,#232685,#232686,#232687,#232688,#232689,
#232690,#232691,#232692,#232693,#232694,#232695,#232696,#232697,#232698,
#232699,#232700,#232701,#232702,#232703,#232704,#232705,#232706,#232707,
#232708,#232709,#232710,#232711,#232712,#232713,#232714,#232715,#232716,
#232717,#232718,#232719,#232720,#232721,#232722,#232723,#232724,#232725,
#232726,#232727),.UNSPECIFIED.,.F.,.F.,(4,3,3,3,3,3,3,3,3,3,3,3,3,3,3,3,
3,4),(4.33680868994202E-19,4.29652152162623E-5,8.44519107536651E-5,0.000123669830865264,
0.000159788877358329,0.000170558847912636,0.000181218775907175,0.000181960046452412,
0.000214460062643658,0.000244755726198798,0.000255838271868947,0.000258503253867581,
0.000261084955178759,0.000289370476647833,0.000301101325502008,0.000321109510663633,
0.000331113603244445,0.000341117695825257),.UNSPECIFIED.);
#5055=B_SPLINE_CURVE_WITH_KNOTS('',3,(#232729,#232730,#232731,#232732,#232733,
#232734,#232735,#232736,#232737,#232738,#232739,#232740,#232741,#232742,
#232743,#232744,#232745,#232746,#232747,#232748,#232749,#232750,#232751,
#232752,#232753,#232754,#232755,#232756,#232757,#232758,#232759,#232760,
#232761,#232762,#232763,#232764,#232765,#232766,#232767,#232768,#232769,
#232770,#232771,#232772,#232773,#232774,#232775,#232776,#232777,#232778,
#232779,#232780),.UNSPECIFIED.,.F.,.F.,(4,3,3,3,3,3,3,3,3,3,3,3,3,3,3,3,
3,4),(3.03576608295941E-18,4.30706237878269E-5,8.47417087712909E-5,0.000124159989208148,
0.000160467076293277,0.000170998382116696,0.000182414994733774,0.00021374797764587,
0.000242415955903288,0.000256497573175043,0.000259169422895616,0.000261757777312422,
0.000289965130403097,0.000301877270772906,0.000321937017503147,0.000326951954185708,
0.000334474359209549,0.000341996764233389),.UNSPECIFIED.);
#5056=B_SPLINE_CURVE_WITH_KNOTS('',3,(#232781,#232782,#232783,#232784,#232785,
#232786,#232787,#232788,#232789,#232790,#232791,#232792,#232793,#232794,
#232795,#232796,#232797,#232798,#232799,#232800,#232801,#232802,#232803,
#232804,#232805,#232806,#232807,#232808,#232809,#232810,#232811,#232812,
#232813,#232814,#232815,#232816,#232817,#232818,#232819,#232820,#232821,
#232822,#232823,#232824,#232825,#232826,#232827,#232828,#232829,#232830,
#232831,#232832),.UNSPECIFIED.,.F.,.F.,(4,3,3,3,3,3,3,3,3,3,3,3,3,3,3,3,
3,4),(0.,2.58457451702089E-5,4.25394446196088E-5,6.46659869687252E-5,7.57292581432834E-5,
8.12608937305625E-5,8.26438026273823E-5,8.67925293178416E-5,0.000116015624427369,
0.000130188793976762,0.000151886926306223,0.000161963651211283,0.000162735992470953,
0.000173585058635683,0.000212487880460468,0.000255238173510466,0.000301397761144727,
0.000347170117271358),.UNSPECIFIED.);
#5057=B_SPLINE_CURVE_WITH_KNOTS('',3,(#232834,#232835,#232836,#232837,#232838,
#232839,#232840,#232841,#232842,#232843,#232844,#232845,#232846,#232847,
#232848,#232849,#232850,#232851,#232852,#232853,#232854,#232855,#232856,
#232857,#232858,#232859,#232860,#232861,#232862,#232863,#232864,#232865,
#232866,#232867,#232868,#232869,#232870,#232871,#232872,#232873,#232874,
#232875,#232876,#232877,#232878,#232879),.UNSPECIFIED.,.F.,.F.,(4,3,3,3,
3,3,3,3,3,3,3,3,3,3,3,4),(0.,2.57218161987217E-5,4.21568322567636E-5,6.45873314616907E-5,
7.58025810641543E-5,8.14102058653861E-5,8.28121120656941E-5,8.70178306666179E-5,
0.000116081955658106,0.000130526745999927,0.000162394111022036,0.000174035661333236,
0.000213138396955684,0.000256116935428608,0.000302406662847822,0.000348071322666479),
 .UNSPECIFIED.);
#5058=B_SPLINE_CURVE_WITH_KNOTS('',3,(#232880,#232881,#232882,#232883,#232884,
#232885,#232886,#232887,#232888,#232889,#232890,#232891,#232892,#232893,
#232894,#232895,#232896,#232897,#232898,#232899,#232900,#232901,#232902,
#232903,#232904,#232905,#232906,#232907,#232908,#232909,#232910,#232911,
#232912,#232913,#232914,#232915,#232916,#232917,#232918,#232919,#232920,
#232921,#232922,#232923,#232924,#232925,#232926,#232927,#232928,#232929,
#232930,#232931),.UNSPECIFIED.,.F.,.F.,(4,3,3,3,3,3,3,3,3,3,3,3,3,3,3,3,
3,4),(0.,4.29652152151169E-5,8.4451910752229E-5,0.000123669830864283,0.000159788877358467,
0.000170558847912639,0.000181218775907178,0.000181960046452411,0.00021446006264415,
0.000244755726200223,0.00025583827186895,0.000258503253867585,0.000261084955178762,
0.000289370476646099,0.000301101325502012,0.000321109510663636,0.000331113603244449,
0.000341117695825261),.UNSPECIFIED.);
#5059=B_SPLINE_CURVE_WITH_KNOTS('',3,(#232933,#232934,#232935,#232936,#232937,
#232938,#232939,#232940,#232941,#232942,#232943,#232944,#232945,#232946,
#232947,#232948,#232949,#232950,#232951,#232952,#232953,#232954,#232955,
#232956,#232957,#232958,#232959,#232960,#232961,#232962,#232963,#232964,
#232965,#232966,#232967,#232968,#232969,#232970,#232971,#232972,#232973,
#232974,#232975,#232976,#232977,#232978,#232979,#232980,#232981,#232982,
#232983,#232984),.UNSPECIFIED.,.F.,.F.,(4,3,3,3,3,3,3,3,3,3,3,3,3,3,3,3,
3,4),(0.,4.30706237873135E-5,8.47417087702485E-5,0.000124159989206487,0.000160467076290862,
0.000170998382116686,0.000182414994733771,0.000213747977645862,0.000242415955902801,
0.000256497573175037,0.000259169422895611,0.000261757777312416,0.000289965130403939,
0.000301877270772903,0.000321937017503146,0.000326951954185706,0.000334474359209548,
0.000341996764233389),.UNSPECIFIED.);
#5060=B_SPLINE_CURVE_WITH_KNOTS('',3,(#232985,#232986,#232987,#232988,#232989,
#232990,#232991,#232992,#232993,#232994,#232995,#232996,#232997,#232998,
#232999,#233000,#233001,#233002,#233003,#233004,#233005,#233006,#233007,
#233008,#233009,#233010,#233011,#233012,#233013,#233014,#233015,#233016,
#233017,#233018,#233019,#233020,#233021,#233022,#233023,#233024,#233025,
#233026,#233027,#233028,#233029,#233030,#233031,#233032,#233033,#233034,
#233035,#233036),.UNSPECIFIED.,.F.,.F.,(4,3,3,3,3,3,3,3,3,3,3,3,3,3,3,3,
3,4),(0.,2.58457451693913E-5,4.2539444619546E-5,6.46659869686941E-5,7.57292581432681E-5,
8.12608937305551E-5,8.26438026273769E-5,8.67925293178422E-5,0.000116015624427399,
0.000130188793976763,0.000151886926306224,0.000161963651211272,0.000162735992470954,
0.000173585058635684,0.000212487880460446,0.000255238173511253,0.000301397761147859,
0.000347170117271368),.UNSPECIFIED.);
#5061=B_SPLINE_CURVE_WITH_KNOTS('',3,(#233038,#233039,#233040,#233041,#233042,
#233043,#233044,#233045,#233046,#233047,#233048,#233049,#233050,#233051,
#233052,#233053,#233054,#233055,#233056,#233057,#233058,#233059,#233060,
#233061,#233062,#233063,#233064,#233065,#233066,#233067,#233068,#233069,
#233070,#233071,#233072,#233073,#233074,#233075,#233076,#233077,#233078,
#233079,#233080,#233081,#233082,#233083),.UNSPECIFIED.,.F.,.F.,(4,3,3,3,
3,3,3,3,3,3,3,3,3,3,3,4),(0.,2.57218161993301E-5,4.21568322567844E-5,6.45873314617024E-5,
7.58025810641613E-5,8.14102058653908E-5,8.28121120656982E-5,8.70178306666203E-5,
0.000116081955658652,0.00013052674599993,0.000162394111022054,0.000174035661333241,
0.00021313839696057,0.000256116935438433,0.000302406662863314,0.000348071322666482),
 .UNSPECIFIED.);
#5062=B_SPLINE_CURVE_WITH_KNOTS('',3,(#233084,#233085,#233086,#233087,#233088,
#233089,#233090,#233091,#233092,#233093,#233094,#233095,#233096,#233097,
#233098,#233099,#233100,#233101,#233102,#233103,#233104,#233105,#233106,
#233107,#233108,#233109,#233110,#233111,#233112,#233113,#233114,#233115,
#233116,#233117,#233118,#233119,#233120,#233121,#233122,#233123,#233124,
#233125,#233126,#233127,#233128,#233129,#233130,#233131,#233132,#233133,
#233134,#233135),.UNSPECIFIED.,.F.,.F.,(4,3,3,3,3,3,3,3,3,3,3,3,3,3,3,3,
3,4),(0.,4.29652152133293E-5,8.44519107489887E-5,0.000123669830859642,0.000159788877352289,
0.000170558847912625,0.000181218775907164,0.000181960046452431,0.000214460062644072,
0.000244755726200207,0.000255838271868938,0.000258503253867573,0.00026108495517875,
0.000289370476647827,0.000301101325502001,0.000321109510663626,0.000331113603244438,
0.000341117695825251),.UNSPECIFIED.);
#5063=B_SPLINE_CURVE_WITH_KNOTS('',3,(#233137,#233138,#233139,#233140,#233141,
#233142,#233143,#233144,#233145,#233146,#233147,#233148,#233149,#233150,
#233151,#233152,#233153,#233154,#233155,#233156,#233157,#233158,#233159,
#233160,#233161,#233162,#233163,#233164,#233165,#233166,#233167,#233168,
#233169,#233170,#233171,#233172,#233173,#233174,#233175,#233176,#233177,
#233178,#233179,#233180,#233181,#233182,#233183,#233184,#233185,#233186,
#233187,#233188),.UNSPECIFIED.,.F.,.F.,(4,3,3,3,3,3,3,3,3,3,3,3,3,3,3,3,
3,4),(0.,4.30706237846825E-5,8.47417087656643E-5,0.000124159989200225,0.000160467076282839,
0.000170998382116685,0.000182414994733771,0.00021374797764586,0.000242415955903785,
0.000256497573175036,0.000259169422895609,0.000261757777312415,0.000289965130404008,
0.000301877270772901,0.000321937017503144,0.000326951954185705,0.000334474359209546,
0.000341996764233387),.UNSPECIFIED.);
#5064=B_SPLINE_CURVE_WITH_KNOTS('',3,(#233189,#233190,#233191,#233192,#233193,
#233194,#233195,#233196,#233197,#233198,#233199,#233200,#233201,#233202,
#233203,#233204,#233205,#233206,#233207,#233208,#233209,#233210,#233211,
#233212,#233213,#233214,#233215,#233216,#233217,#233218,#233219,#233220,
#233221,#233222,#233223,#233224,#233225,#233226,#233227,#233228,#233229,
#233230,#233231,#233232,#233233,#233234,#233235,#233236,#233237,#233238,
#233239,#233240),.UNSPECIFIED.,.F.,.F.,(4,3,3,3,3,3,3,3,3,3,3,3,3,3,3,3,
3,4),(0.,2.58457451681982E-5,4.25394446197375E-5,6.46659869687881E-5,7.57292581433134E-5,
8.1260893730576E-5,8.26438026273917E-5,8.67925293178387E-5,0.000116015624428111,
0.000130188793976758,0.000151886926306218,0.000161963651211279,0.000162735992470948,
0.000173585058635677,0.000212487880463093,0.000255238173516002,0.000301397761153951,
0.000347170117271371),.UNSPECIFIED.);
#5065=B_SPLINE_CURVE_WITH_KNOTS('',3,(#233242,#233243,#233244,#233245,#233246,
#233247,#233248,#233249,#233250,#233251,#233252,#233253,#233254,#233255,
#233256,#233257,#233258,#233259,#233260,#233261,#233262,#233263,#233264,
#233265,#233266,#233267,#233268,#233269,#233270,#233271,#233272,#233273,
#233274,#233275,#233276,#233277,#233278,#233279,#233280,#233281,#233282,
#233283,#233284,#233285,#233286,#233287),.UNSPECIFIED.,.F.,.F.,(4,3,3,3,
3,3,3,3,3,3,3,3,3,3,3,4),(0.,2.57218161997734E-5,4.21568322567237E-5,6.45873314616717E-5,
7.58025810641458E-5,8.14102058653828E-5,8.2812112065692E-5,8.70178306666198E-5,
0.00011608195565779,0.00013052674599993,0.000162394111022048,0.00017403566133324,
0.000213138396958063,0.00025611693543337,0.000302406662855231,0.000348071322666498),
 .UNSPECIFIED.);
#5066=B_SPLINE_CURVE_WITH_KNOTS('',3,(#233288,#233289,#233290,#233291,#233292,
#233293,#233294,#233295,#233296,#233297,#233298,#233299,#233300,#233301,
#233302,#233303,#233304,#233305,#233306,#233307,#233308,#233309,#233310,
#233311,#233312,#233313,#233314,#233315,#233316,#233317,#233318,#233319,
#233320,#233321,#233322,#233323,#233324,#233325,#233326,#233327,#233328,
#233329,#233330,#233331,#233332,#233333,#233334,#233335,#233336,#233337,
#233338,#233339),.UNSPECIFIED.,.F.,.F.,(4,3,3,3,3,3,3,3,3,3,3,3,3,3,3,3,
3,4),(0.,4.29652152152899E-5,8.44519107520695E-5,0.000123669830863396,0.000159788877356221,
0.000170558847912629,0.000181218775907169,0.00018196004645238,0.000214460062643359,
0.000244755726197827,0.000255838271868951,0.000258503253867586,0.000261084955178764,
0.000289370476648966,0.000301101325502019,0.000321109510663646,0.00033111360324446,
0.000341117695825274),.UNSPECIFIED.);
#5067=B_SPLINE_CURVE_WITH_KNOTS('',3,(#233341,#233342,#233343,#233344,#233345,
#233346,#233347,#233348,#233349,#233350,#233351,#233352,#233353,#233354,
#233355,#233356,#233357,#233358,#233359,#233360,#233361,#233362,#233363,
#233364,#233365,#233366,#233367,#233368,#233369,#233370,#233371,#233372,
#233373,#233374,#233375,#233376,#233377,#233378,#233379,#233380,#233381,
#233382,#233383,#233384,#233385,#233386,#233387,#233388,#233389,#233390,
#233391,#233392),.UNSPECIFIED.,.F.,.F.,(4,3,3,3,3,3,3,3,3,3,3,3,3,3,3,3,
3,4),(4.33680868994202E-19,4.30706237891753E-5,8.47417087736514E-5,0.000124159989211244,
0.00016046707629719,0.000170998382116694,0.000182414994733769,0.000213747977645867,
0.000242415955902945,0.00025649757317504,0.000259169422895614,0.000261757777312419,
0.000289965130403412,0.000301877270772903,0.000321937017503145,0.000326951954185705,
0.000334474359209546,0.000341996764233387),.UNSPECIFIED.);
#5068=B_SPLINE_CURVE_WITH_KNOTS('',3,(#233393,#233394,#233395,#233396,#233397,
#233398,#233399,#233400,#233401,#233402,#233403,#233404,#233405,#233406,
#233407,#233408,#233409,#233410,#233411,#233412,#233413,#233414,#233415,
#233416,#233417,#233418,#233419,#233420,#233421,#233422,#233423,#233424,
#233425,#233426,#233427,#233428,#233429,#233430,#233431,#233432,#233433,
#233434,#233435,#233436,#233437,#233438,#233439,#233440,#233441,#233442,
#233443,#233444),.UNSPECIFIED.,.F.,.F.,(4,3,3,3,3,3,3,3,3,3,3,3,3,3,3,3,
3,4),(0.,2.58457451678341E-5,4.25394446195883E-5,6.46659869687171E-5,7.57292581432815E-5,
8.12608937305636E-5,8.26438026273842E-5,8.67925293178458E-5,0.000116015624426969,
0.000130188793976769,0.00015188692630623,0.000161963651211286,0.000162735992470961,
0.000173585058635692,0.000212487880461625,0.000255238173512158,0.00030139776114569,
0.000347170117271384),.UNSPECIFIED.);
#5069=B_SPLINE_CURVE_WITH_KNOTS('',3,(#233446,#233447,#233448,#233449,#233450,
#233451,#233452,#233453,#233454,#233455,#233456,#233457,#233458,#233459,
#233460,#233461,#233462,#233463,#233464,#233465,#233466,#233467,#233468,
#233469,#233470,#233471,#233472,#233473,#233474,#233475,#233476,#233477,
#233478,#233479,#233480,#233481,#233482,#233483,#233484,#233485,#233486,
#233487,#233488,#233489,#233490,#233491),.UNSPECIFIED.,.F.,.F.,(4,3,3,3,
3,3,3,3,3,3,3,3,3,3,3,4),(0.,2.57218161985664E-5,4.21568322568204E-5,6.45873314617178E-5,
7.58025810641665E-5,8.14102058653908E-5,8.28121120656969E-5,8.70178306666152E-5,
0.000116081955657799,0.000130526745999923,0.000162394111022031,0.00017403566133323,
0.00021313839695763,0.000256116935432652,0.000302406662854616,0.00034807132266646),
 .UNSPECIFIED.);
#5070=B_SPLINE_CURVE_WITH_KNOTS('',3,(#233492,#233493,#233494,#233495,#233496,
#233497,#233498,#233499,#233500,#233501,#233502,#233503,#233504,#233505,
#233506,#233507,#233508,#233509,#233510,#233511,#233512,#233513,#233514,
#233515,#233516,#233517,#233518,#233519,#233520,#233521,#233522,#233523,
#233524,#233525,#233526,#233527,#233528,#233529,#233530,#233531,#233532,
#233533,#233534,#233535,#233536,#233537,#233538,#233539,#233540,#233541,
#233542,#233543),.UNSPECIFIED.,.F.,.F.,(4,3,3,3,3,3,3,3,3,3,3,3,3,3,3,3,
3,4),(4.33680868994202E-19,4.2965215218658E-5,8.44519107577739E-5,0.000123669830870734,
0.000159788877365064,0.000170558847912629,0.000181218775907169,0.000181960046452411,
0.000214460062643825,0.000244755726198647,0.000255838271868945,0.00025850325386758,
0.000261084955178758,0.000289370476647757,0.00030110132550201,0.000321109510663636,
0.000331113603244449,0.000341117695825262),.UNSPECIFIED.);
#5071=B_SPLINE_CURVE_WITH_KNOTS('',3,(#233545,#233546,#233547,#233548,#233549,
#233550,#233551,#233552,#233553,#233554,#233555,#233556,#233557,#233558,
#233559,#233560,#233561,#233562,#233563,#233564,#233565,#233566,#233567,
#233568,#233569,#233570,#233571,#233572,#233573,#233574,#233575,#233576,
#233577,#233578,#233579,#233580,#233581,#233582,#233583,#233584,#233585,
#233586,#233587,#233588,#233589,#233590,#233591,#233592,#233593,#233594,
#233595,#233596),.UNSPECIFIED.,.F.,.F.,(4,3,3,3,3,3,3,3,3,3,3,3,3,3,3,3,
3,4),(0.,4.30706237853674E-5,8.47417087668512E-5,0.000124159989201798,0.000160467076284875,
0.000170998382116698,0.00018241499473378,0.000213747977645872,0.00024241595590339,
0.000256497573175045,0.000259169422895618,0.000261757777312424,0.000289965130402989,
0.000301877270772908,0.00032193701750315,0.00032695195418571,0.000334474359209551,
0.000341996764233392),.UNSPECIFIED.);
#5072=B_SPLINE_CURVE_WITH_KNOTS('',3,(#233597,#233598,#233599,#233600,#233601,
#233602,#233603,#233604,#233605,#233606,#233607,#233608,#233609,#233610,
#233611,#233612,#233613,#233614,#233615,#233616,#233617,#233618,#233619,
#233620,#233621,#233622,#233623,#233624,#233625,#233626,#233627,#233628,
#233629,#233630,#233631,#233632,#233633,#233634,#233635,#233636,#233637,
#233638,#233639,#233640,#233641,#233642,#233643,#233644,#233645,#233646,
#233647,#233648),.UNSPECIFIED.,.F.,.F.,(4,3,3,3,3,3,3,3,3,3,3,3,3,3,3,3,
3,4),(0.,2.5845745169787E-5,4.25394446194455E-5,6.46659869686411E-5,7.57292581432389E-5,
8.12608937305378E-5,8.26438026273625E-5,8.67925293178367E-5,0.000116015624427309,
0.000130188793976755,0.000151886926306214,0.000161963651211279,0.000162735992470944,
0.000173585058635673,0.000212487880458767,0.000255238173506756,0.000301397761138237,
0.000347170117271364),.UNSPECIFIED.);
#5073=B_SPLINE_CURVE_WITH_KNOTS('',3,(#233650,#233651,#233652,#233653,#233654,
#233655,#233656,#233657,#233658,#233659,#233660,#233661,#233662,#233663,
#233664,#233665,#233666,#233667,#233668,#233669,#233670,#233671,#233672,
#233673,#233674,#233675,#233676,#233677,#233678,#233679,#233680,#233681,
#233682,#233683,#233684,#233685,#233686,#233687,#233688,#233689,#233690,
#233691,#233692,#233693,#233694,#233695),.UNSPECIFIED.,.F.,.F.,(4,3,3,3,
3,3,3,3,3,3,3,3,3,3,3,4),(0.,2.57218161994861E-5,4.21568322567979E-5,6.45873314617086E-5,
7.5802581064164E-5,8.14102058653917E-5,8.28121120656986E-5,8.70178306666193E-5,
0.000116081955658953,0.000130526745999929,0.000162394111022036,0.000174035661333239,
0.000213138396959787,0.000256116935436981,0.000302406662861451,0.000348071322666494),
 .UNSPECIFIED.);
#5074=B_SPLINE_CURVE_WITH_KNOTS('',3,(#233696,#233697,#233698,#233699,#233700,
#233701,#233702,#233703,#233704,#233705,#233706,#233707,#233708,#233709,
#233710,#233711,#233712,#233713,#233714,#233715,#233716,#233717,#233718,
#233719,#233720,#233721,#233722,#233723,#233724,#233725,#233726,#233727,
#233728,#233729,#233730,#233731,#233732,#233733,#233734,#233735,#233736,
#233737,#233738,#233739,#233740,#233741,#233742,#233743,#233744,#233745,
#233746,#233747),.UNSPECIFIED.,.F.,.F.,(4,3,3,3,3,3,3,3,3,3,3,3,3,3,3,3,
3,4),(0.,4.29652152170427E-5,8.44519107551245E-5,0.000123669830867409,0.000159788877361216,
0.000170558847912622,0.000181218775907161,0.000181960046452394,0.000214460062643908,
0.000244755726199335,0.00025583827186894,0.000258503253867575,0.000261084955178753,
0.000289370476646841,0.000301101325502006,0.000321109510663632,0.000331113603244446,
0.000341117695825259),.UNSPECIFIED.);
#5075=B_SPLINE_CURVE_WITH_KNOTS('',3,(#233749,#233750,#233751,#233752,#233753,
#233754,#233755,#233756,#233757,#233758,#233759,#233760,#233761,#233762,
#233763,#233764,#233765,#233766,#233767,#233768,#233769,#233770,#233771,
#233772,#233773,#233774,#233775,#233776,#233777,#233778,#233779,#233780,
#233781,#233782,#233783,#233784,#233785,#233786,#233787,#233788,#233789,
#233790,#233791,#233792,#233793,#233794,#233795,#233796,#233797,#233798,
#233799,#233800),.UNSPECIFIED.,.F.,.F.,(4,3,3,3,3,3,3,3,3,3,3,3,3,3,3,3,
3,4),(1.73472347597681E-18,4.30706237846257E-5,8.47417087654249E-5,0.000124159989199596,
0.000160467076281756,0.000170998382116706,0.000182414994733789,0.000213747977645876,
0.000242415955904062,0.000256497573175046,0.000259169422895619,0.000261757777312425,
0.000289965130401927,0.000301877270772905,0.000321937017503146,0.000326951954185706,
0.000334474359209546,0.000341996764233386),.UNSPECIFIED.);
#5076=B_SPLINE_CURVE_WITH_KNOTS('',3,(#233801,#233802,#233803,#233804,#233805,
#233806,#233807,#233808,#233809,#233810,#233811,#233812,#233813,#233814,
#233815,#233816,#233817,#233818,#233819,#233820,#233821,#233822,#233823,
#233824,#233825,#233826,#233827,#233828,#233829,#233830,#233831,#233832,
#233833,#233834,#233835,#233836,#233837,#233838,#233839,#233840,#233841,
#233842,#233843,#233844,#233845,#233846,#233847,#233848,#233849,#233850,
#233851,#233852),.UNSPECIFIED.,.F.,.F.,(4,3,3,3,3,3,3,3,3,3,3,3,3,3,3,3,
3,4),(0.,2.58457451679675E-5,4.25394446195623E-5,6.46659869687017E-5,7.57292581432714E-5,
8.12608937305563E-5,8.26438026273775E-5,8.67925293178412E-5,0.000116015624427185,
0.000130188793976762,0.000151886926306222,0.000161963651211282,0.000162735992470952,
0.000173585058635682,0.000212487880461526,0.000255238173513458,0.000301397761151195,
0.000347170117271365),.UNSPECIFIED.);
#5077=B_SPLINE_CURVE_WITH_KNOTS('',3,(#233854,#233855,#233856,#233857,#233858,
#233859,#233860,#233861,#233862,#233863,#233864,#233865,#233866,#233867,
#233868,#233869,#233870,#233871,#233872,#233873,#233874,#233875,#233876,
#233877,#233878,#233879,#233880,#233881,#233882,#233883,#233884,#233885,
#233886,#233887,#233888,#233889,#233890,#233891,#233892,#233893,#233894,
#233895,#233896,#233897,#233898,#233899),.UNSPECIFIED.,.F.,.F.,(4,3,3,3,
3,3,3,3,3,3,3,3,3,3,3,4),(0.,2.57218162002627E-5,4.21568322568371E-5,6.45873314617265E-5,
7.58025810641712E-5,8.14102058653936E-5,8.28121120656992E-5,8.70178306666159E-5,
0.000116081955658511,0.000130526745999924,0.000162394111022038,0.000174035661333232,
0.000213138396959335,0.00025611693543601,0.000302406662859656,0.000348071322666466),
 .UNSPECIFIED.);
#5078=B_SPLINE_CURVE_WITH_KNOTS('',3,(#233900,#233901,#233902,#233903,#233904,
#233905,#233906,#233907,#233908,#233909,#233910,#233911,#233912,#233913,
#233914,#233915,#233916,#233917,#233918,#233919,#233920,#233921,#233922,
#233923,#233924,#233925,#233926,#233927,#233928,#233929,#233930,#233931,
#233932,#233933,#233934,#233935,#233936,#233937,#233938,#233939,#233940,
#233941,#233942,#233943,#233944,#233945,#233946,#233947,#233948,#233949,
#233950,#233951),.UNSPECIFIED.,.F.,.F.,(4,3,3,3,3,3,3,3,3,3,3,3,3,3,3,3,
3,4),(0.,4.29652152182024E-5,8.44519107564933E-5,0.00012366983086809,0.000159788877360639,
0.000170558847912628,0.000181218775907167,0.000181960046452403,0.000214460062643301,
0.000244755726197727,0.000255838271868942,0.000258503253867577,0.000261084955178754,
0.00028937047664789,0.000301101325502005,0.000321109510663631,0.000331113603244444,
0.000341117695825256),.UNSPECIFIED.);
#5079=B_SPLINE_CURVE_WITH_KNOTS('',3,(#233953,#233954,#233955,#233956,#233957,
#233958,#233959,#233960,#233961,#233962,#233963,#233964,#233965,#233966,
#233967,#233968,#233969,#233970,#233971,#233972,#233973,#233974,#233975,
#233976,#233977,#233978,#233979,#233980,#233981,#233982,#233983,#233984,
#233985,#233986,#233987,#233988,#233989,#233990,#233991,#233992,#233993,
#233994,#233995,#233996,#233997,#233998,#233999,#234000,#234001,#234002,
#234003,#234004),.UNSPECIFIED.,.F.,.F.,(4,3,3,3,3,3,3,3,3,3,3,3,3,3,3,3,
3,4),(1.30104260698261E-18,4.30706237875003E-5,8.47417087704618E-5,0.000124159989206612,
0.00016046707629077,0.000170998382116696,0.00018241499473378,0.000213747977645868,
0.000242415955902669,0.00025649757317504,0.000259169422895613,0.000261757777312418,
0.00028996513040356,0.000301877270772901,0.000321937017503142,0.000326951954185702,
0.000334474359209543,0.000341996764233383),.UNSPECIFIED.);
#5080=B_SPLINE_CURVE_WITH_KNOTS('',3,(#234005,#234006,#234007,#234008,#234009,
#234010,#234011,#234012,#234013,#234014,#234015,#234016,#234017,#234018,
#234019,#234020,#234021,#234022,#234023,#234024,#234025,#234026,#234027,
#234028,#234029,#234030,#234031,#234032,#234033,#234034,#234035,#234036,
#234037,#234038,#234039,#234040,#234041,#234042,#234043,#234044,#234045,
#234046,#234047,#234048,#234049,#234050,#234051,#234052,#234053,#234054,
#234055,#234056),.UNSPECIFIED.,.F.,.F.,(4,3,3,3,3,3,3,3,3,3,3,3,3,3,3,3,
3,4),(0.,2.58457451671873E-5,4.25394446196736E-5,6.46659869687558E-5,7.5729258143297E-5,
8.12608937305675E-5,8.26438026273852E-5,8.67925293178381E-5,0.000116015624426789,
0.000130188793976757,0.000151886926306217,0.000161963651211268,0.000162735992470946,
0.000173585058635676,0.000212487880462401,0.000255238173514613,0.000301397761151736,
0.000347170117271366),.UNSPECIFIED.);
#5081=B_SPLINE_CURVE_WITH_KNOTS('',3,(#234058,#234059,#234060,#234061,#234062,
#234063,#234064,#234065,#234066,#234067,#234068,#234069,#234070,#234071,
#234072,#234073,#234074,#234075,#234076,#234077,#234078,#234079,#234080,
#234081,#234082,#234083,#234084,#234085,#234086,#234087,#234088,#234089,
#234090,#234091,#234092,#234093,#234094,#234095,#234096,#234097,#234098,
#234099,#234100,#234101,#234102,#234103),.UNSPECIFIED.,.F.,.F.,(4,3,3,3,
3,3,3,3,3,3,3,3,3,3,3,4),(0.,2.57218161987729E-5,4.21568322568131E-5,6.45873314617148E-5,
7.58025810641656E-5,8.1410205865391E-5,8.28121120656974E-5,8.70178306666164E-5,
0.000116081955658176,0.000130526745999925,0.000162394111022042,0.000174035661333233,
0.000213138396957878,0.00025611693543317,0.000302406662855509,0.000348071322666435),
 .UNSPECIFIED.);
#5082=B_SPLINE_CURVE_WITH_KNOTS('',3,(#234104,#234105,#234106,#234107,#234108,
#234109,#234110,#234111,#234112,#234113,#234114,#234115,#234116,#234117,
#234118,#234119,#234120,#234121,#234122,#234123,#234124,#234125,#234126,
#234127,#234128,#234129,#234130,#234131,#234132,#234133,#234134,#234135,
#234136,#234137,#234138,#234139,#234140,#234141,#234142,#234143,#234144,
#234145,#234146,#234147,#234148,#234149,#234150,#234151,#234152,#234153,
#234154,#234155),.UNSPECIFIED.,.F.,.F.,(4,3,3,3,3,3,3,3,3,3,3,3,3,3,3,3,
3,4),(0.,4.29652152218646E-5,8.44519107628296E-5,0.000123669830876734,0.000159788877371542,
0.000170558847912634,0.000181218775907173,0.000181960046452415,0.00021446006264388,
0.000244755726199356,0.000255838271868947,0.000258503253867581,0.000261084955178759,
0.000289370476646635,0.000301101325502009,0.000321109510663634,0.000331113603244447,
0.000341117695825259),.UNSPECIFIED.);
#5083=B_SPLINE_CURVE_WITH_KNOTS('',3,(#234157,#234158,#234159,#234160,#234161,
#234162,#234163,#234164,#234165,#234166,#234167,#234168,#234169,#234170,
#234171,#234172,#234173,#234174,#234175,#234176,#234177,#234178,#234179,
#234180,#234181,#234182,#234183,#234184,#234185,#234186,#234187,#234188,
#234189,#234190,#234191,#234192,#234193,#234194,#234195,#234196,#234197,
#234198,#234199,#234200,#234201,#234202,#234203,#234204,#234205,#234206,
#234207,#234208),.UNSPECIFIED.,.F.,.F.,(4,3,3,3,3,3,3,3,3,3,3,3,3,3,3,3,
3,4),(8.68445263380243E-18,4.30706237867881E-5,8.47417087695995E-5,0.000124159989206084,
0.000160467076290811,0.000170998382116702,0.000182414994733779,0.000213747977645876,
0.000242415955903851,0.000256497573175051,0.000259169422895625,0.00026175777731243,
0.00028996513040331,0.000301877270772915,0.000321937017503158,0.000326951954185719,
0.00033447435920956,0.000341996764233401),.UNSPECIFIED.);
#5084=B_SPLINE_CURVE_WITH_KNOTS('',3,(#234209,#234210,#234211,#234212,#234213,
#234214,#234215,#234216,#234217,#234218,#234219,#234220,#234221,#234222,
#234223,#234224,#234225,#234226,#234227,#234228,#234229,#234230,#234231,
#234232,#234233,#234234,#234235,#234236,#234237,#234238,#234239,#234240,
#234241,#234242,#234243,#234244,#234245,#234246,#234247,#234248,#234249,
#234250,#234251,#234252,#234253,#234254,#234255,#234256,#234257,#234258,
#234259,#234260),.UNSPECIFIED.,.F.,.F.,(4,3,3,3,3,3,3,3,3,3,3,3,3,3,3,3,
3,4),(0.,2.58457451680534E-5,4.25394446195252E-5,6.46659869686818E-5,7.57292581432601E-5,
8.12608937305493E-5,8.26438026273716E-5,8.67925293178384E-5,0.000116015624427207,
0.000130188793976758,0.000151886926306217,0.000161963651211286,0.000162735992470947,
0.000173585058635677,0.00021248788045977,0.000255238173509542,0.000301397761144293,
0.000347170117271369),.UNSPECIFIED.);
#5085=B_SPLINE_CURVE_WITH_KNOTS('',3,(#234262,#234263,#234264,#234265,#234266,
#234267,#234268,#234269,#234270,#234271,#234272,#234273,#234274,#234275,
#234276,#234277,#234278,#234279,#234280,#234281,#234282,#234283,#234284,
#234285,#234286,#234287,#234288,#234289,#234290,#234291,#234292,#234293,
#234294,#234295,#234296,#234297,#234298,#234299,#234300,#234301,#234302,
#234303,#234304,#234305,#234306,#234307),.UNSPECIFIED.,.F.,.F.,(4,3,3,3,
3,3,3,3,3,3,3,3,3,3,3,4),(3.46944695195361E-18,2.57218162013466E-5,4.21568322567922E-5,
6.45873314617082E-5,7.58025810641662E-5,8.14102058653952E-5,8.28121120657025E-5,
8.70178306666242E-5,0.0001160819556593,0.000130526745999935,0.000162394111022058,
0.000174035661333245,0.00021313839695979,0.000256116935436838,0.000302406662860849,
0.000348071322666457),.UNSPECIFIED.);
#5086=B_SPLINE_CURVE_WITH_KNOTS('',3,(#234308,#234309,#234310,#234311,#234312,
#234313,#234314,#234315,#234316,#234317,#234318,#234319,#234320,#234321,
#234322,#234323,#234324,#234325,#234326,#234327,#234328,#234329,#234330,
#234331,#234332,#234333,#234334,#234335,#234336,#234337,#234338,#234339,
#234340,#234341,#234342,#234343,#234344,#234345,#234346,#234347,#234348,
#234349,#234350,#234351,#234352,#234353,#234354,#234355,#234356,#234357,
#234358,#234359),.UNSPECIFIED.,.F.,.F.,(4,3,3,3,3,3,3,3,3,3,3,3,3,3,3,3,
3,4),(0.,4.29652152143574E-5,8.44519107509678E-5,0.000123669830862744,0.000159788877356808,
0.000170558847912645,0.000181218775907184,0.000181960046452413,0.00021446006264388,
0.000244755726199279,0.000255838271868959,0.000258503253867594,0.000261084955178771,
0.000289370476647778,0.000301101325502022,0.000321109510663648,0.00033111360324446,
0.000341117695825273),.UNSPECIFIED.);
#5087=B_SPLINE_CURVE_WITH_KNOTS('',3,(#234361,#234362,#234363,#234364,#234365,
#234366,#234367,#234368,#234369,#234370,#234371,#234372,#234373,#234374,
#234375,#234376,#234377,#234378,#234379,#234380,#234381,#234382,#234383,
#234384,#234385,#234386,#234387,#234388,#234389,#234390,#234391,#234392,
#234393,#234394,#234395,#234396,#234397,#234398,#234399,#234400,#234401,
#234402,#234403,#234404,#234405,#234406,#234407,#234408,#234409,#234410,
#234411,#234412),.UNSPECIFIED.,.F.,.F.,(4,3,3,3,3,3,3,3,3,3,3,3,3,3,3,3,
3,4),(0.,4.30706237877896E-5,8.47417087711211E-5,0.000124159989207682,0.000160467076292507,
0.000170998382116696,0.000182414994733788,0.000213747977645869,0.000242415955903998,
0.000256497573175042,0.000259169422895615,0.000261757777312421,0.000289965130402697,
0.000301877270772904,0.000321937017503146,0.000326951954185707,0.000334474359209547,
0.000341996764233388),.UNSPECIFIED.);
#5088=B_SPLINE_CURVE_WITH_KNOTS('',3,(#234413,#234414,#234415,#234416,#234417,
#234418,#234419,#234420,#234421,#234422,#234423,#234424,#234425,#234426,
#234427,#234428,#234429,#234430,#234431,#234432,#234433,#234434,#234435,
#234436,#234437,#234438,#234439,#234440,#234441,#234442,#234443,#234444,
#234445,#234446,#234447,#234448,#234449,#234450,#234451,#234452,#234453,
#234454,#234455,#234456,#234457,#234458,#234459,#234460,#234461,#234462,
#234463,#234464),.UNSPECIFIED.,.F.,.F.,(4,3,3,3,3,3,3,3,3,3,3,3,3,3,3,3,
3,4),(0.,2.58457451671327E-5,4.25394446196085E-5,6.46659869687207E-5,7.57292581432768E-5,
8.12608937305548E-5,8.26438026273743E-5,8.67925293178329E-5,0.000116015624427058,
0.000130188793976749,0.000151886926306208,0.000161963651211277,0.000162735992470937,
0.000173585058635666,0.000212487880460147,0.000255238173510913,0.000301397761147941,
0.000347170117271348),.UNSPECIFIED.);
#5089=B_SPLINE_CURVE_WITH_KNOTS('',3,(#234466,#234467,#234468,#234469,#234470,
#234471,#234472,#234473,#234474,#234475,#234476,#234477,#234478,#234479,
#234480,#234481,#234482,#234483,#234484,#234485,#234486,#234487,#234488,
#234489,#234490,#234491,#234492,#234493,#234494,#234495,#234496,#234497,
#234498,#234499,#234500,#234501,#234502,#234503,#234504,#234505,#234506,
#234507,#234508,#234509,#234510,#234511),.UNSPECIFIED.,.F.,.F.,(4,3,3,3,
3,3,3,3,3,3,3,3,3,3,3,4),(1.73472347597681E-18,2.57218162001682E-5,4.21568322567692E-5,
6.45873314616974E-5,7.58025810641615E-5,8.14102058653936E-5,8.28121120657016E-5,
8.70178306666256E-5,0.000116081955658883,0.000130526745999938,0.000162394111022063,
0.00017403566133325,0.000213138396957746,0.000256116935432846,0.000302406662854858,
0.000348071322666484),.UNSPECIFIED.);
#5090=B_SPLINE_CURVE_WITH_KNOTS('',3,(#234512,#234513,#234514,#234515,#234516,
#234517,#234518,#234519,#234520,#234521,#234522,#234523,#234524,#234525,
#234526,#234527,#234528,#234529,#234530,#234531,#234532,#234533,#234534,
#234535,#234536,#234537,#234538,#234539,#234540,#234541,#234542,#234543,
#234544,#234545,#234546,#234547,#234548,#234549,#234550,#234551,#234552,
#234553,#234554,#234555,#234556,#234557,#234558,#234559,#234560,#234561,
#234562,#234563),.UNSPECIFIED.,.F.,.F.,(4,3,3,3,3,3,3,3,3,3,3,3,3,3,3,3,
3,4),(4.33680868994202E-19,4.29652152122471E-5,8.44519107475262E-5,0.000123669830858404,
0.000159788877351739,0.000170558847912622,0.000181218775907162,0.000181960046452396,
0.000214460062643998,0.00024475572619965,0.000255838271868939,0.000258503253867574,
0.000261084955178751,0.000289370476647007,0.000301101325502003,0.000321109510663629,
0.000331113603244442,0.000341117695825255),.UNSPECIFIED.);
#5091=B_SPLINE_CURVE_WITH_KNOTS('',3,(#234565,#234566,#234567,#234568,#234569,
#234570,#234571,#234572,#234573,#234574,#234575,#234576,#234577,#234578,
#234579,#234580,#234581,#234582,#234583,#234584,#234585,#234586,#234587,
#234588,#234589,#234590,#234591,#234592,#234593,#234594,#234595,#234596,
#234597,#234598,#234599,#234600,#234601,#234602,#234603,#234604,#234605,
#234606,#234607,#234608,#234609,#234610,#234611,#234612,#234613,#234614,
#234615,#234616),.UNSPECIFIED.,.F.,.F.,(4,3,3,3,3,3,3,3,3,3,3,3,3,3,3,3,
3,4),(4.33680868994202E-19,4.30706237874098E-5,8.47417087703705E-5,0.000124159989206565,
0.000160467076290862,0.000170998382116692,0.000182414994733768,0.000213747977645868,
0.000242415955904643,0.000256497573175044,0.000259169422895618,0.000261757777312423,
0.000289965130402133,0.000301877270772906,0.000321937017503148,0.000326951954185708,
0.000334474359209549,0.000341996764233389),.UNSPECIFIED.);
#5092=B_SPLINE_CURVE_WITH_KNOTS('',3,(#234617,#234618,#234619,#234620,#234621,
#234622,#234623,#234624,#234625,#234626,#234627,#234628,#234629,#234630,
#234631,#234632,#234633,#234634,#234635,#234636,#234637,#234638,#234639,
#234640,#234641,#234642,#234643,#234644,#234645,#234646,#234647,#234648,
#234649,#234650,#234651,#234652,#234653,#234654,#234655,#234656,#234657,
#234658,#234659,#234660,#234661,#234662,#234663,#234664,#234665,#234666,
#234667,#234668),.UNSPECIFIED.,.F.,.F.,(4,3,3,3,3,3,3,3,3,3,3,3,3,3,3,3,
3,4),(0.,2.58457451681173E-5,4.25394446196654E-5,6.46659869687525E-5,7.5729258143296E-5,
8.12608937305678E-5,8.26438026273857E-5,8.67925293178395E-5,0.00011601562442695,
0.000130188793976759,0.000151886926306219,0.000161963651211275,0.000162735992470949,
0.000173585058635679,0.00021248788045979,0.00025523817350832,0.000301397761139514,
0.000347170117271359),.UNSPECIFIED.);
#5093=B_SPLINE_CURVE_WITH_KNOTS('',3,(#234670,#234671,#234672,#234673,#234674,
#234675,#234676,#234677,#234678,#234679,#234680,#234681,#234682,#234683,
#234684,#234685,#234686,#234687,#234688,#234689,#234690,#234691,#234692,
#234693,#234694,#234695,#234696,#234697,#234698,#234699,#234700,#234701,
#234702,#234703,#234704,#234705,#234706,#234707,#234708,#234709,#234710,
#234711,#234712,#234713,#234714,#234715),.UNSPECIFIED.,.F.,.F.,(4,3,3,3,
3,3,3,3,3,3,3,3,3,3,3,4),(1.73472347597681E-18,2.57218161991517E-5,4.21568322568403E-5,
6.45873314617371E-5,7.58025810641855E-5,8.14102058654097E-5,8.28121120657157E-5,
8.70178306666339E-5,0.000116081955658399,0.00013052674599995,0.000162394111022071,
0.000174035661333266,0.000213138396959586,0.000256116935436441,0.000302406662860196,
0.000348071322666516),.UNSPECIFIED.);
#5094=B_SPLINE_CURVE_WITH_KNOTS('',3,(#234716,#234717,#234718,#234719,#234720,
#234721,#234722,#234723,#234724,#234725,#234726,#234727,#234728,#234729,
#234730,#234731,#234732,#234733,#234734,#234735,#234736,#234737,#234738,
#234739,#234740,#234741,#234742,#234743,#234744,#234745,#234746,#234747,
#234748,#234749,#234750,#234751,#234752,#234753,#234754,#234755,#234756,
#234757,#234758,#234759,#234760,#234761,#234762,#234763,#234764,#234765,
#234766,#234767),.UNSPECIFIED.,.F.,.F.,(4,3,3,3,3,3,3,3,3,3,3,3,3,3,3,3,
3,4),(4.33680868994202E-19,4.29652152179851E-5,8.44519107563622E-5,0.000123669830868358,
0.000159788877361452,0.000170558847912632,0.000181218775907171,0.00018196004645241,
0.000214460062643803,0.00024475572619926,0.000255838271868948,0.000258503253867583,
0.000261084955178761,0.000289370476647563,0.000301101325502013,0.000321109510663639,
0.000331113603244452,0.000341117695825265),.UNSPECIFIED.);
#5095=B_SPLINE_CURVE_WITH_KNOTS('',3,(#234769,#234770,#234771,#234772,#234773,
#234774,#234775,#234776,#234777,#234778,#234779,#234780,#234781,#234782,
#234783,#234784,#234785,#234786,#234787,#234788,#234789,#234790,#234791,
#234792,#234793,#234794,#234795,#234796,#234797,#234798,#234799,#234800,
#234801,#234802,#234803,#234804,#234805,#234806,#234807,#234808,#234809,
#234810,#234811,#234812,#234813,#234814,#234815,#234816,#234817,#234818,
#234819,#234820),.UNSPECIFIED.,.F.,.F.,(4,3,3,3,3,3,3,3,3,3,3,3,3,3,3,3,
3,4),(0.,4.30706237861595E-5,8.4741708768375E-5,0.000124159989204126,0.000160467076288123,
0.000170998382116677,0.000182414994733771,0.000213747977645853,0.000242415955903301,
0.000256497573175029,0.000259169422895603,0.000261757777312408,0.000289965130402838,
0.000301877270772894,0.000321937017503137,0.000326951954185698,0.000334474359209539,
0.000341996764233381),.UNSPECIFIED.);
#5096=B_SPLINE_CURVE_WITH_KNOTS('',3,(#234821,#234822,#234823,#234824,#234825,
#234826,#234827,#234828,#234829,#234830,#234831,#234832,#234833,#234834,
#234835,#234836,#234837,#234838,#234839,#234840,#234841,#234842,#234843,
#234844,#234845,#234846,#234847,#234848,#234849,#234850,#234851,#234852,
#234853,#234854,#234855,#234856,#234857,#234858,#234859,#234860,#234861,
#234862,#234863,#234864,#234865,#234866,#234867,#234868,#234869,#234870,
#234871,#234872),.UNSPECIFIED.,.F.,.F.,(4,3,3,3,3,3,3,3,3,3,3,3,3,3,3,3,
3,4),(0.,2.58457451685323E-5,4.25394446196102E-5,6.46659869687251E-5,7.57292581432825E-5,
8.12608937305612E-5,8.26438026273809E-5,8.679252931784E-5,0.000116015624427535,
0.00013018879397676,0.00015188692630622,0.000161963651211282,0.00016273599247095,
0.00017358505863568,0.000212487880460561,0.000255238173511503,0.000301397761148276,
0.000347170117271346),.UNSPECIFIED.);
#5097=B_SPLINE_CURVE_WITH_KNOTS('',3,(#234874,#234875,#234876,#234877,#234878,
#234879,#234880,#234881,#234882,#234883,#234884,#234885,#234886,#234887,
#234888,#234889,#234890,#234891,#234892,#234893,#234894,#234895,#234896,
#234897,#234898,#234899,#234900,#234901,#234902,#234903,#234904,#234905,
#234906,#234907,#234908,#234909,#234910,#234911,#234912,#234913,#234914,
#234915,#234916,#234917,#234918,#234919),.UNSPECIFIED.,.F.,.F.,(4,3,3,3,
3,3,3,3,3,3,3,3,3,3,3,4),(5.48877349820787E-19,2.57218161988899E-5,4.21568322568674E-5,
6.45873314617467E-5,7.58025810641863E-5,8.14102058654061E-5,8.28121120657111E-5,
8.70178306666259E-5,0.000116081955658109,0.000130526745999939,0.000162394111022064,
0.000174035661333251,0.000213138396957216,0.000256116935431698,0.000302406662852769,
0.000348071322666503),.UNSPECIFIED.);
#5098=B_SPLINE_CURVE_WITH_KNOTS('',3,(#234920,#234921,#234922,#234923,#234924,
#234925,#234926,#234927,#234928,#234929,#234930,#234931,#234932,#234933,
#234934,#234935,#234936,#234937,#234938,#234939,#234940,#234941,#234942,
#234943,#234944,#234945,#234946,#234947,#234948,#234949,#234950,#234951,
#234952,#234953,#234954,#234955,#234956,#234957,#234958,#234959,#234960,
#234961,#234962,#234963,#234964,#234965,#234966,#234967,#234968,#234969,
#234970,#234971),.UNSPECIFIED.,.F.,.F.,(4,3,3,3,3,3,3,3,3,3,3,3,3,3,3,3,
3,4),(0.,4.29652152139708E-5,8.44519107499793E-5,0.000123669830860699,0.000159788877353224,
0.00017055884791263,0.000181218775907169,0.000181960046452404,0.000214460062643146,
0.000244755726197271,0.000255838271868945,0.00025850325386758,0.000261084955178757,
0.000289370476648699,0.000301101325502009,0.000321109510663634,0.000331113603244447,
0.00034111769582526),.UNSPECIFIED.);
#5099=B_SPLINE_CURVE_WITH_KNOTS('',3,(#234973,#234974,#234975,#234976,#234977,
#234978,#234979,#234980,#234981,#234982,#234983,#234984,#234985,#234986,
#234987,#234988,#234989,#234990,#234991,#234992,#234993,#234994,#234995,
#234996,#234997,#234998,#234999,#235000,#235001,#235002,#235003,#235004,
#235005,#235006,#235007,#235008,#235009,#235010,#235011,#235012,#235013,
#235014,#235015,#235016,#235017,#235018,#235019,#235020,#235021,#235022,
#235023,#235024),.UNSPECIFIED.,.F.,.F.,(4,3,3,3,3,3,3,3,3,3,3,3,3,3,3,3,
3,4),(9.85133562538035E-18,4.30706237881605E-5,8.47417087718283E-5,0.000124159989208858,
0.0001604670762942,0.000170998382116695,0.000182414994733785,0.000213747977645867,
0.000242415955903381,0.000256497573175038,0.000259169422895612,0.000261757777312417,
0.00028996513040321,0.000301877270772899,0.00032193701750314,0.000326951954185701,
0.000334474359209541,0.000341996764233381),.UNSPECIFIED.);
#5100=B_SPLINE_CURVE_WITH_KNOTS('',3,(#235025,#235026,#235027,#235028,#235029,
#235030,#235031,#235032,#235033,#235034,#235035,#235036,#235037,#235038,
#235039,#235040,#235041,#235042,#235043,#235044,#235045,#235046,#235047,
#235048,#235049,#235050,#235051,#235052,#235053,#235054,#235055,#235056,
#235057,#235058,#235059,#235060,#235061,#235062,#235063,#235064,#235065,
#235066,#235067,#235068,#235069,#235070,#235071,#235072,#235073,#235074,
#235075,#235076),.UNSPECIFIED.,.F.,.F.,(4,3,3,3,3,3,3,3,3,3,3,3,3,3,3,3,
3,4),(0.,2.58457451672615E-5,4.25394446195262E-5,6.46659869686852E-5,7.57292581432647E-5,
8.12608937305545E-5,8.26438026273769E-5,8.67925293178442E-5,0.0001160156244269,
0.000130188793976766,0.000151886926306227,0.000161963651211279,0.000162735992470958,
0.000173585058635688,0.000212487880460214,0.000255238173510026,0.000301397761144323,
0.000347170117271377),.UNSPECIFIED.);
#5101=B_SPLINE_CURVE_WITH_KNOTS('',3,(#235078,#235079,#235080,#235081,#235082,
#235083,#235084,#235085,#235086,#235087,#235088,#235089,#235090,#235091,
#235092,#235093,#235094,#235095,#235096,#235097,#235098,#235099,#235100,
#235101,#235102,#235103,#235104,#235105,#235106,#235107,#235108,#235109,
#235110,#235111,#235112,#235113,#235114,#235115,#235116,#235117,#235118,
#235119,#235120,#235121,#235122,#235123),.UNSPECIFIED.,.F.,.F.,(4,3,3,3,
3,3,3,3,3,3,3,3,3,3,3,4),(8.67361737988403E-19,2.57218161987776E-5,4.21568322567847E-5,
6.45873314617043E-5,7.58025810641641E-5,8.1410205865394E-5,8.28121120657015E-5,
8.7017830666624E-5,0.000116081955658135,0.000130526745999932,0.000162394111022062,
0.000174035661333239,0.000213138396959045,0.000256116935435313,0.000302406662858188,
0.000348071322666484),.UNSPECIFIED.);
#5102=B_SPLINE_CURVE_WITH_KNOTS('',3,(#235124,#235125,#235126,#235127,#235128,
#235129,#235130,#235131,#235132,#235133,#235134,#235135,#235136,#235137,
#235138,#235139,#235140,#235141,#235142,#235143,#235144,#235145,#235146,
#235147,#235148,#235149,#235150,#235151,#235152,#235153,#235154,#235155,
#235156,#235157,#235158,#235159,#235160,#235161,#235162,#235163,#235164,
#235165,#235166,#235167,#235168,#235169,#235170,#235171,#235172,#235173,
#235174,#235175),.UNSPECIFIED.,.F.,.F.,(4,3,3,3,3,3,3,3,3,3,3,3,3,3,3,3,
3,4),(0.,4.29652152157613E-5,8.44519107527578E-5,0.000123669830863927,0.000159788877356499,
0.000170558847912623,0.000181218775907163,0.000181960046452398,0.000214460062643952,
0.00024475572619948,0.000255838271868942,0.000258503253867577,0.000261084955178755,
0.000289370476647228,0.000301101325502008,0.000321109510663634,0.000331113603244447,
0.000341117695825261),.UNSPECIFIED.);
#5103=B_SPLINE_CURVE_WITH_KNOTS('',3,(#235177,#235178,#235179,#235180,#235181,
#235182,#235183,#235184,#235185,#235186,#235187,#235188,#235189,#235190,
#235191,#235192,#235193,#235194,#235195,#235196,#235197,#235198,#235199,
#235200,#235201,#235202,#235203,#235204,#235205,#235206,#235207,#235208,
#235209,#235210,#235211,#235212,#235213,#235214,#235215,#235216,#235217,
#235218,#235219,#235220,#235221,#235222,#235223,#235224,#235225,#235226,
#235227,#235228),.UNSPECIFIED.,.F.,.F.,(4,3,3,3,3,3,3,3,3,3,3,3,3,3,3,3,
3,4),(3.03576608295941E-18,4.30706237875898E-5,8.47417087709076E-5,0.000124159989207655,
0.000160467076292736,0.000170998382116693,0.000182414994733774,0.000213747977645865,
0.000242415955903445,0.000256497573175038,0.000259169422895611,0.000261757777312417,
0.000289965130403454,0.0003018772707729,0.000321937017503142,0.000326951954185703,
0.000334474359209543,0.000341996764233384),.UNSPECIFIED.);
#5104=B_SPLINE_CURVE_WITH_KNOTS('',3,(#235229,#235230,#235231,#235232,#235233,
#235234,#235235,#235236,#235237,#235238,#235239,#235240,#235241,#235242,
#235243,#235244,#235245,#235246,#235247,#235248,#235249,#235250,#235251,
#235252,#235253,#235254,#235255,#235256,#235257,#235258,#235259,#235260,
#235261,#235262,#235263,#235264,#235265,#235266,#235267,#235268,#235269,
#235270,#235271,#235272,#235273,#235274,#235275,#235276,#235277,#235278,
#235279,#235280),.UNSPECIFIED.,.F.,.F.,(4,3,3,3,3,3,3,3,3,3,3,3,3,3,3,3,
3,4),(0.,2.58457451669222E-5,4.25394446196541E-5,6.46659869687471E-5,7.57292581432935E-5,
8.12608937305668E-5,8.26438026273851E-5,8.679252931784E-5,0.000116015624426832,
0.00013018879397676,0.00015188692630622,0.000161963651211278,0.00016273599247095,
0.00017358505863568,0.00021248788046056,0.000255238173511179,0.000301397761147054,
0.000347170117271364),.UNSPECIFIED.);
#5105=B_SPLINE_CURVE_WITH_KNOTS('',3,(#235282,#235283,#235284,#235285,#235286,
#235287,#235288,#235289,#235290,#235291,#235292,#235293,#235294,#235295,
#235296,#235297,#235298,#235299,#235300,#235301,#235302,#235303,#235304,
#235305,#235306,#235307,#235308,#235309,#235310,#235311,#235312,#235313,
#235314,#235315,#235316,#235317,#235318,#235319,#235320,#235321,#235322,
#235323,#235324,#235325,#235326,#235327),.UNSPECIFIED.,.F.,.F.,(4,3,3,3,
3,3,3,3,3,3,3,3,3,3,3,4),(0.,2.57218162009012E-5,4.21568322567646E-5,6.45873314616925E-5,
7.58025810641564E-5,8.14102058653884E-5,8.28121120656964E-5,8.70178306666204E-5,
0.000116081955658897,0.000130526745999931,0.000162394111022045,0.000174035661333241,
0.000213138396957201,0.000256116935431684,0.000302406662852778,0.000348071322666473),
 .UNSPECIFIED.);
#5106=B_SPLINE_CURVE_WITH_KNOTS('',3,(#235328,#235329,#235330,#235331,#235332,
#235333,#235334,#235335,#235336,#235337,#235338,#235339,#235340,#235341,
#235342,#235343,#235344,#235345,#235346,#235347,#235348,#235349,#235350,
#235351,#235352,#235353,#235354,#235355,#235356,#235357,#235358,#235359,
#235360,#235361,#235362,#235363,#235364,#235365,#235366,#235367,#235368,
#235369,#235370,#235371,#235372,#235373,#235374,#235375,#235376,#235377,
#235378,#235379),.UNSPECIFIED.,.F.,.F.,(4,3,3,3,3,3,3,3,3,3,3,3,3,3,3,3,
3,4),(0.,4.29652152152673E-5,8.44519107521068E-5,0.000123669830863404,0.000159788877356394,
0.000170558847912628,0.000181218775907168,0.000181960046452405,0.000214460062643706,
0.000244755726199078,0.000255838271868944,0.000258503253867578,0.000261084955178756,
0.000289370476647239,0.000301101325502007,0.000321109510663633,0.000331113603244446,
0.000341117695825259),.UNSPECIFIED.);
#5107=B_SPLINE_CURVE_WITH_KNOTS('',3,(#235381,#235382,#235383,#235384,#235385,
#235386,#235387,#235388,#235389,#235390,#235391,#235392,#235393,#235394,
#235395,#235396,#235397,#235398,#235399,#235400,#235401,#235402,#235403,
#235404,#235405,#235406,#235407,#235408,#235409,#235410,#235411,#235412,
#235413,#235414,#235415,#235416,#235417,#235418,#235419,#235420,#235421,
#235422,#235423,#235424,#235425,#235426,#235427,#235428,#235429,#235430,
#235431,#235432),.UNSPECIFIED.,.F.,.F.,(4,3,3,3,3,3,3,3,3,3,3,3,3,3,3,3,
3,4),(3.03576608295941E-18,4.30706237872071E-5,8.474170877004E-5,0.00012415998920614,
0.000160467076290401,0.000170998382116706,0.000182414994733797,0.000213747977645878,
0.000242415955903907,0.000256497573175049,0.000259169422895622,0.000261757777312428,
0.000289965130403662,0.00030187727077291,0.000321937017503151,0.000326951954185711,
0.000334474359209552,0.000341996764233392),.UNSPECIFIED.);
#5108=B_SPLINE_CURVE_WITH_KNOTS('',3,(#235433,#235434,#235435,#235436,#235437,
#235438,#235439,#235440,#235441,#235442,#235443,#235444,#235445,#235446,
#235447,#235448,#235449,#235450,#235451,#235452,#235453,#235454,#235455,
#235456,#235457,#235458,#235459,#235460,#235461,#235462,#235463,#235464,
#235465,#235466,#235467,#235468,#235469,#235470,#235471,#235472,#235473,
#235474,#235475,#235476,#235477,#235478,#235479,#235480,#235481,#235482,
#235483,#235484),.UNSPECIFIED.,.F.,.F.,(4,3,3,3,3,3,3,3,3,3,3,3,3,3,3,3,
3,4),(0.,2.58457451681574E-5,4.2539444619624E-5,6.46659869687327E-5,7.5729258143287E-5,
8.12608937305642E-5,8.26438026273834E-5,8.67925293178413E-5,0.000116015624427458,
0.000130188793976762,0.000151886926306222,0.000161963651211265,0.000162735992470952,
0.000173585058635683,0.000212487880461666,0.000255238173513071,0.000301397761149064,
0.000347170117271372),.UNSPECIFIED.);
#5109=B_SPLINE_CURVE_WITH_KNOTS('',3,(#235486,#235487,#235488,#235489,#235490,
#235491,#235492,#235493,#235494,#235495,#235496,#235497,#235498,#235499,
#235500,#235501,#235502,#235503,#235504,#235505,#235506,#235507,#235508,
#235509,#235510,#235511,#235512,#235513,#235514,#235515,#235516,#235517,
#235518,#235519,#235520,#235521,#235522,#235523,#235524,#235525,#235526,
#235527,#235528,#235529,#235530,#235531),.UNSPECIFIED.,.F.,.F.,(4,3,3,3,
3,3,3,3,3,3,3,3,3,3,3,4),(0.,2.57218161989481E-5,4.21568322568538E-5,6.45873314617329E-5,
7.58025810641724E-5,8.14102058653922E-5,8.28121120656971E-5,8.7017830666612E-5,
0.000116081955658189,0.000130526745999918,0.000162394111022038,0.000174035661333224,
0.000213138396958885,0.000256116935435022,0.000302406662857814,0.00034807132266645),
 .UNSPECIFIED.);
#5110=B_SPLINE_CURVE_WITH_KNOTS('',3,(#235532,#235533,#235534,#235535,#235536,
#235537,#235538,#235539,#235540,#235541,#235542,#235543,#235544,#235545,
#235546,#235547,#235548,#235549,#235550,#235551,#235552,#235553,#235554,
#235555,#235556,#235557,#235558,#235559,#235560,#235561,#235562,#235563,
#235564,#235565,#235566,#235567,#235568,#235569,#235570,#235571,#235572,
#235573,#235574,#235575,#235576,#235577,#235578,#235579,#235580,#235581,
#235582,#235583),.UNSPECIFIED.,.F.,.F.,(4,3,3,3,3,3,3,3,3,3,3,3,3,3,3,3,
3,4),(4.33680868994202E-19,4.2965215221666E-5,8.44519107623575E-5,0.000123669830875747,
0.000159788877369812,0.000170558847912634,0.000181218775907173,0.000181960046452406,
0.00021446006264371,0.00024475572619867,0.000255838271868942,0.000258503253867577,
0.000261084955178754,0.000289370476647226,0.000301101325502002,0.000321109510663626,
0.000331113603244438,0.00034111769582525),.UNSPECIFIED.);
#5111=B_SPLINE_CURVE_WITH_KNOTS('',3,(#235585,#235586,#235587,#235588,#235589,
#235590,#235591,#235592,#235593,#235594,#235595,#235596,#235597,#235598,
#235599,#235600,#235601,#235602,#235603,#235604,#235605,#235606,#235607,
#235608,#235609,#235610,#235611,#235612,#235613,#235614,#235615,#235616,
#235617,#235618,#235619,#235620,#235621,#235622,#235623,#235624,#235625,
#235626,#235627,#235628,#235629,#235630,#235631,#235632,#235633,#235634,
#235635,#235636),.UNSPECIFIED.,.F.,.F.,(4,3,3,3,3,3,3,3,3,3,3,3,3,3,3,3,
3,4),(0.,4.30706237877873E-5,8.47417087710622E-5,0.000124159989207586,0.000160467076292239,
0.000170998382116696,0.000182414994733785,0.000213747977645869,0.000242415955902956,
0.000256497573175042,0.000259169422895616,0.000261757777312421,0.000289965130403431,
0.000301877270772905,0.000321937017503147,0.000326951954185708,0.000334474359209548,
0.000341996764233389),.UNSPECIFIED.);
#5112=B_SPLINE_CURVE_WITH_KNOTS('',3,(#235637,#235638,#235639,#235640,#235641,
#235642,#235643,#235644,#235645,#235646,#235647,#235648,#235649,#235650,
#235651,#235652,#235653,#235654,#235655,#235656,#235657,#235658,#235659,
#235660,#235661,#235662,#235663,#235664,#235665,#235666,#235667,#235668,
#235669,#235670,#235671,#235672,#235673,#235674,#235675,#235676,#235677,
#235678,#235679,#235680,#235681,#235682,#235683,#235684,#235685,#235686,
#235687,#235688),.UNSPECIFIED.,.F.,.F.,(4,3,3,3,3,3,3,3,3,3,3,3,3,3,3,3,
3,4),(0.,2.58457451676357E-5,4.25394446196733E-5,6.46659869687554E-5,7.57292581432964E-5,
8.1260893730567E-5,8.26438026273846E-5,8.67925293178375E-5,0.000116015624426936,
0.000130188793976756,0.000151886926306216,0.000161963651211277,0.000162735992470945,
0.000173585058635675,0.000212487880461714,0.000255238173514346,0.00030139776115405,
0.000347170117271358),.UNSPECIFIED.);
#5113=B_SPLINE_CURVE_WITH_KNOTS('',3,(#235690,#235691,#235692,#235693,#235694,
#235695,#235696,#235697,#235698,#235699,#235700,#235701,#235702,#235703,
#235704,#235705,#235706,#235707,#235708,#235709,#235710,#235711,#235712,
#235713,#235714,#235715,#235716,#235717,#235718,#235719,#235720,#235721,
#235722,#235723,#235724,#235725,#235726,#235727,#235728,#235729,#235730,
#235731,#235732,#235733,#235734,#235735),.UNSPECIFIED.,.F.,.F.,(4,3,3,3,
3,3,3,3,3,3,3,3,3,3,3,4),(3.46944695195361E-18,2.57218162006677E-5,4.2156832256807E-5,
6.45873314617123E-5,7.5802581064165E-5,8.14102058653913E-5,8.28121120656978E-5,
8.70178306666176E-5,0.000116081955659339,0.000130526745999925,0.000162394111022045,
0.000174035661333232,0.000213138396960436,0.000256116935438212,0.000302406662863133,
0.00034807132266646),.UNSPECIFIED.);
#5114=B_SPLINE_CURVE_WITH_KNOTS('',3,(#235736,#235737,#235738,#235739,#235740,
#235741,#235742,#235743,#235744,#235745,#235746,#235747,#235748,#235749,
#235750,#235751,#235752,#235753,#235754,#235755,#235756,#235757,#235758,
#235759,#235760,#235761,#235762,#235763,#235764,#235765,#235766,#235767,
#235768,#235769,#235770,#235771,#235772,#235773,#235774,#235775,#235776,
#235777,#235778,#235779,#235780,#235781,#235782,#235783,#235784,#235785,
#235786,#235787),.UNSPECIFIED.,.F.,.F.,(4,3,3,3,3,3,3,3,3,3,3,3,3,3,3,3,
3,4),(0.,4.29652152160775E-5,8.44519107533754E-5,0.000123669830864951,0.00015978887735793,
0.000170558847912619,0.000181218775907159,0.000181960046452398,0.000214460062643413,
0.000244755726197593,0.000255838271868937,0.000258503253867572,0.00026108495517875,
0.000289370476648662,0.000301101325502003,0.000321109510663629,0.000331113603244443,
0.000341117695825256),.UNSPECIFIED.);
#5115=B_SPLINE_CURVE_WITH_KNOTS('',3,(#235789,#235790,#235791,#235792,#235793,
#235794,#235795,#235796,#235797,#235798,#235799,#235800,#235801,#235802,
#235803,#235804,#235805,#235806,#235807,#235808,#235809,#235810,#235811,
#235812,#235813,#235814,#235815,#235816,#235817,#235818,#235819,#235820,
#235821,#235822,#235823,#235824,#235825,#235826,#235827,#235828,#235829,
#235830,#235831,#235832,#235833,#235834,#235835,#235836,#235837,#235838,
#235839,#235840),.UNSPECIFIED.,.F.,.F.,(4,3,3,3,3,3,3,3,3,3,3,3,3,3,3,3,
3,4),(0.,4.30706237882173E-5,8.47417087719784E-5,0.000124159989209114,0.000160467076294534,
0.000170998382116702,0.000182414994733779,0.000213747977645877,0.0002424159559042,
0.000256497573175052,0.000259169422895626,0.000261757777312431,0.000289965130403038,
0.000301877270772917,0.00032193701750316,0.000326951954185721,0.000334474359209562,
0.000341996764233403),.UNSPECIFIED.);
#5116=B_SPLINE_CURVE_WITH_KNOTS('',3,(#235841,#235842,#235843,#235844,#235845,
#235846,#235847,#235848,#235849,#235850,#235851,#235852,#235853,#235854,
#235855,#235856,#235857,#235858,#235859,#235860,#235861,#235862,#235863,
#235864,#235865,#235866,#235867,#235868,#235869,#235870,#235871,#235872,
#235873,#235874,#235875,#235876,#235877,#235878,#235879,#235880,#235881,
#235882,#235883,#235884,#235885,#235886,#235887,#235888,#235889,#235890,
#235891,#235892),.UNSPECIFIED.,.F.,.F.,(4,3,3,3,3,3,3,3,3,3,3,3,3,3,3,3,
3,4),(0.,2.58457451679575E-5,4.25394446196678E-5,6.46659869687542E-5,7.57292581432974E-5,
8.1260893730569E-5,8.26438026273869E-5,8.67925293178406E-5,0.000116015624427285,
0.000130188793976761,0.000151886926306221,0.000161963651211261,0.000162735992470951,
0.000173585058635681,0.000212487880457631,0.000255238173503925,0.000301397761132213,
0.000347170117271364),.UNSPECIFIED.);
#5117=B_SPLINE_CURVE_WITH_KNOTS('',3,(#235894,#235895,#235896,#235897,#235898,
#235899,#235900,#235901,#235902,#235903,#235904,#235905,#235906,#235907,
#235908,#235909,#235910,#235911,#235912,#235913,#235914,#235915,#235916,
#235917,#235918,#235919,#235920,#235921,#235922,#235923,#235924,#235925,
#235926,#235927,#235928,#235929,#235930,#235931,#235932,#235933,#235934,
#235935,#235936,#235937,#235938,#235939),.UNSPECIFIED.,.F.,.F.,(4,3,3,3,
3,3,3,3,3,3,3,3,3,3,3,4),(0.,2.57218161982287E-5,4.21568322568021E-5,6.45873314617112E-5,
7.58025810641658E-5,8.1410205865393E-5,8.28121120656999E-5,8.70178306666203E-5,
0.000116081955657987,0.00013052674599993,0.000162394111022054,0.000174035661333241,
0.000213138396958526,0.000256116935434306,0.00030240666285673,0.000348071322666488),
 .UNSPECIFIED.);
#5118=B_SPLINE_CURVE_WITH_KNOTS('',3,(#235940,#235941,#235942,#235943,#235944,
#235945,#235946,#235947,#235948,#235949,#235950,#235951,#235952,#235953,
#235954,#235955,#235956,#235957,#235958,#235959,#235960,#235961,#235962,
#235963,#235964,#235965,#235966,#235967,#235968,#235969,#235970,#235971,
#235972,#235973,#235974,#235975,#235976,#235977,#235978,#235979,#235980,
#235981,#235982,#235983,#235984,#235985,#235986,#235987,#235988,#235989,
#235990,#235991),.UNSPECIFIED.,.F.,.F.,(4,3,3,3,3,3,3,3,3,3,3,3,3,3,3,3,
3,4),(2.16840434497101E-18,4.29652152152268E-5,8.44519107520661E-5,0.00012366983086337,
0.000159788877356357,0.000170558847912644,0.000181218775907183,0.000181960046452433,
0.000214460062643565,0.000244755726198341,0.000255838271868955,0.00025850325386759,
0.000261084955178768,0.000289370476647945,0.000301101325502017,0.000321109510663642,
0.000331113603244455,0.000341117695825267),.UNSPECIFIED.);
#5119=B_SPLINE_CURVE_WITH_KNOTS('',3,(#235993,#235994,#235995,#235996,#235997,
#235998,#235999,#236000,#236001,#236002,#236003,#236004,#236005,#236006,
#236007,#236008,#236009,#236010,#236011,#236012,#236013,#236014,#236015,
#236016,#236017,#236018,#236019,#236020,#236021,#236022,#236023,#236024,
#236025,#236026,#236027,#236028,#236029,#236030,#236031,#236032,#236033,
#236034,#236035,#236036,#236037,#236038,#236039,#236040,#236041,#236042,
#236043,#236044),.UNSPECIFIED.,.F.,.F.,(4,3,3,3,3,3,3,3,3,3,3,3,3,3,3,3,
3,4),(0.,4.30706237861587E-5,8.47417087681614E-5,0.000124159989203496,0.000160467076286933,
0.000170998382116704,0.000182414994733766,0.000213747977645876,0.000242415955903066,
0.000256497573175048,0.000259169422895621,0.000261757777312426,0.00028996513040416,
0.000301877270772909,0.00032193701750315,0.000326951954185711,0.000334474359209551,
0.000341996764233392),.UNSPECIFIED.);
#5120=B_SPLINE_CURVE_WITH_KNOTS('',3,(#236045,#236046,#236047,#236048,#236049,
#236050,#236051,#236052,#236053,#236054,#236055,#236056,#236057,#236058,
#236059,#236060,#236061,#236062,#236063,#236064,#236065,#236066,#236067,
#236068,#236069,#236070,#236071,#236072,#236073,#236074,#236075,#236076,
#236077,#236078,#236079,#236080,#236081,#236082,#236083,#236084,#236085,
#236086,#236087,#236088,#236089,#236090,#236091,#236092,#236093,#236094,
#236095,#236096),.UNSPECIFIED.,.F.,.F.,(4,3,3,3,3,3,3,3,3,3,3,3,3,3,3,3,
3,4),(0.,2.58457451684377E-5,4.25394446196284E-5,6.46659869687342E-5,7.57292581432872E-5,
8.12608937305636E-5,8.26438026273828E-5,8.67925293178401E-5,0.000116015624426965,
0.00013018879397676,0.00015188692630622,0.000161963651211263,0.00016273599247095,
0.00017358505863568,0.000212487880458883,0.000255238173506548,0.000301397761136831,
0.00034717011727135),.UNSPECIFIED.);
#5121=B_SPLINE_CURVE_WITH_KNOTS('',3,(#236098,#236099,#236100,#236101,#236102,
#236103,#236104,#236105,#236106,#236107,#236108,#236109,#236110,#236111,
#236112,#236113,#236114,#236115,#236116,#236117,#236118,#236119,#236120,
#236121,#236122,#236123,#236124,#236125,#236126,#236127,#236128,#236129,
#236130,#236131,#236132,#236133,#236134,#236135,#236136,#236137,#236138,
#236139,#236140,#236141,#236142,#236143),.UNSPECIFIED.,.F.,.F.,(4,3,3,3,
3,3,3,3,3,3,3,3,3,3,3,4),(6.95243322195995E-18,2.57218161990052E-5,4.21568322569008E-5,
6.4587331461763E-5,7.58025810641941E-5,8.14102058654096E-5,8.28121120657135E-5,
8.70178306666252E-5,0.000116081955658842,0.000130526745999934,0.000162394111022056,
0.000174035661333243,0.000213138396957983,0.000256116935433331,0.000302406662855623,
0.00034807132266648),.UNSPECIFIED.);
#5122=B_SPLINE_CURVE_WITH_KNOTS('',3,(#236144,#236145,#236146,#236147,#236148,
#236149,#236150,#236151,#236152,#236153,#236154,#236155,#236156,#236157,
#236158,#236159,#236160,#236161,#236162,#236163,#236164,#236165,#236166,
#236167,#236168,#236169,#236170,#236171,#236172,#236173,#236174,#236175,
#236176,#236177,#236178,#236179,#236180,#236181,#236182,#236183,#236184,
#236185,#236186,#236187,#236188,#236189,#236190,#236191,#236192,#236193,
#236194,#236195),.UNSPECIFIED.,.F.,.F.,(4,3,3,3,3,3,3,3,3,3,3,3,3,3,3,3,
3,4),(0.,4.29652152188777E-5,8.44519107579093E-5,0.000123669830870508,0.000159788877364258,
0.000170558847912623,0.000181218775907162,0.000181960046452384,0.00021446006264357,
0.000244755726198643,0.000255838271868934,0.000258503253867569,0.000261084955178746,
0.000289370476649059,0.000301101325501996,0.00032110951066362,0.000331113603244433,
0.000341117695825245),.UNSPECIFIED.);
#5123=B_SPLINE_CURVE_WITH_KNOTS('',3,(#236197,#236198,#236199,#236200,#236201,
#236202,#236203,#236204,#236205,#236206,#236207,#236208,#236209,#236210,
#236211,#236212,#236213,#236214,#236215,#236216,#236217,#236218,#236219,
#236220,#236221,#236222,#236223,#236224,#236225,#236226,#236227,#236228,
#236229,#236230,#236231,#236232,#236233,#236234,#236235,#236236,#236237,
#236238,#236239,#236240,#236241,#236242,#236243,#236244,#236245,#236246,
#236247,#236248),.UNSPECIFIED.,.F.,.F.,(4,3,3,3,3,3,3,3,3,3,3,3,3,3,3,3,
3,4),(0.,4.30706237872035E-5,8.47417087699752E-5,0.000124159989205975,0.00016046707629009,
0.000170998382116686,0.000182414994733785,0.000213747977645861,0.000242415955903207,
0.000256497573175036,0.00025916942289561,0.000261757777312415,0.000289965130403885,
0.000301877270772901,0.000321937017503144,0.000326951954185705,0.000334474359209546,
0.000341996764233387),.UNSPECIFIED.);
#5124=B_SPLINE_CURVE_WITH_KNOTS('',3,(#236249,#236250,#236251,#236252,#236253,
#236254,#236255,#236256,#236257,#236258,#236259,#236260,#236261,#236262,
#236263,#236264,#236265,#236266,#236267,#236268,#236269,#236270,#236271,
#236272,#236273,#236274,#236275,#236276,#236277,#236278,#236279,#236280,
#236281,#236282,#236283,#236284,#236285,#236286,#236287,#236288,#236289,
#236290,#236291,#236292,#236293,#236294,#236295,#236296,#236297,#236298,
#236299,#236300),.UNSPECIFIED.,.F.,.F.,(4,3,3,3,3,3,3,3,3,3,3,3,3,3,3,3,
3,4),(0.,2.58457451676233E-5,4.25394446195383E-5,6.46659869686869E-5,7.57292581432612E-5,
8.12608937305484E-5,8.26438026273701E-5,8.67925293178355E-5,0.000116015624427426,
0.000130188793976753,0.000151886926306212,0.000161963651211271,0.000162735992470942,
0.000173585058635671,0.000212487880461207,0.000255238173513124,0.000301397761151479,
0.00034717011727136),.UNSPECIFIED.);
#5125=B_SPLINE_CURVE_WITH_KNOTS('',3,(#236302,#236303,#236304,#236305,#236306,
#236307,#236308,#236309,#236310,#236311,#236312,#236313,#236314,#236315,
#236316,#236317,#236318,#236319,#236320,#236321,#236322,#236323,#236324,
#236325,#236326,#236327,#236328,#236329,#236330,#236331,#236332,#236333,
#236334,#236335,#236336,#236337,#236338,#236339,#236340,#236341,#236342,
#236343,#236344,#236345,#236346,#236347),.UNSPECIFIED.,.F.,.F.,(4,3,3,3,
3,3,3,3,3,3,3,3,3,3,3,4),(0.,2.57218162000743E-5,4.21568322568328E-5,6.45873314617215E-5,
7.58025810641659E-5,8.14102058653881E-5,8.28121120656936E-5,8.70178306666103E-5,
0.000116081955658848,0.000130526745999915,0.000162394111022043,0.000174035661333221,
0.000213138396961521,0.000256116935440342,0.00030240666286625,0.000348071322666455),
 .UNSPECIFIED.);
#5126=B_SPLINE_CURVE_WITH_KNOTS('',3,(#236348,#236349,#236350,#236351,#236352,
#236353,#236354,#236355,#236356,#236357,#236358,#236359,#236360,#236361,
#236362,#236363,#236364,#236365,#236366,#236367,#236368,#236369,#236370,
#236371,#236372,#236373,#236374,#236375,#236376,#236377,#236378,#236379,
#236380,#236381,#236382,#236383,#236384,#236385,#236386,#236387,#236388,
#236389,#236390,#236391,#236392,#236393,#236394,#236395,#236396,#236397,
#236398,#236399),.UNSPECIFIED.,.F.,.F.,(4,3,3,3,3,3,3,3,3,3,3,3,3,3,3,3,
3,4),(1.30104260698261E-18,4.29652152171682E-5,8.4451910755208E-5,0.000123669830867249,
0.000159788877360641,0.000170558847912643,0.000181218775907182,0.000181960046452421,
0.000214460062643499,0.000244755726198127,0.000255838271868955,0.00025850325386759,
0.000261084955178767,0.000289370476646182,0.000301101325502018,0.000321109510663643,
0.000331113603244455,0.000341117695825268),.UNSPECIFIED.);
#5127=B_SPLINE_CURVE_WITH_KNOTS('',3,(#236401,#236402,#236403,#236404,#236405,
#236406,#236407,#236408,#236409,#236410,#236411,#236412,#236413,#236414,
#236415,#236416,#236417,#236418,#236419,#236420,#236421,#236422,#236423,
#236424,#236425,#236426,#236427,#236428,#236429,#236430,#236431,#236432,
#236433,#236434,#236435,#236436,#236437,#236438,#236439,#236440,#236441,
#236442,#236443,#236444,#236445,#236446,#236447,#236448,#236449,#236450,
#236451,#236452),.UNSPECIFIED.,.F.,.F.,(4,3,3,3,3,3,3,3,3,3,3,3,3,3,3,3,
3,4),(2.60208521396521E-18,4.30706237873492E-5,8.4741708770217E-5,0.000124159989206236,
0.000160467076290362,0.000170998382116704,0.000182414994733796,0.000213747977645875,
0.000242415955902185,0.000256497573175047,0.00025916942289562,0.000261757777312426,
0.000289965130404871,0.000301877270772908,0.000321937017503149,0.00032695195418571,
0.00033447435920955,0.000341996764233391),.UNSPECIFIED.);
#5128=B_SPLINE_CURVE_WITH_KNOTS('',3,(#236453,#236454,#236455,#236456,#236457,
#236458,#236459,#236460,#236461,#236462,#236463,#236464,#236465,#236466,
#236467,#236468,#236469,#236470,#236471,#236472,#236473,#236474,#236475,
#236476,#236477,#236478,#236479,#236480,#236481,#236482,#236483,#236484,
#236485,#236486,#236487,#236488,#236489,#236490,#236491,#236492,#236493,
#236494,#236495,#236496,#236497,#236498,#236499,#236500,#236501,#236502,
#236503,#236504),.UNSPECIFIED.,.F.,.F.,(4,3,3,3,3,3,3,3,3,3,3,3,3,3,3,3,
3,4),(0.,2.58457451673697E-5,4.25394446196103E-5,6.46659869687253E-5,7.57292581432827E-5,
8.12608937305615E-5,8.26438026273812E-5,8.67925293178402E-5,0.000116015624426797,
0.00013018879397676,0.00015188692630622,0.000161963651211268,0.00016273599247095,
0.00017358505863568,0.000212487880460138,0.000255238173509389,0.000301397761142022,
0.000347170117271361),.UNSPECIFIED.);
#5129=B_SPLINE_CURVE_WITH_KNOTS('',3,(#236506,#236507,#236508,#236509,#236510,
#236511,#236512,#236513,#236514,#236515,#236516,#236517,#236518,#236519,
#236520,#236521,#236522,#236523,#236524,#236525,#236526,#236527,#236528,
#236529,#236530,#236531,#236532,#236533,#236534,#236535,#236536,#236537,
#236538,#236539,#236540,#236541,#236542,#236543,#236544,#236545,#236546,
#236547,#236548,#236549,#236550,#236551),.UNSPECIFIED.,.F.,.F.,(4,3,3,3,
3,3,3,3,3,3,3,3,3,3,3,4),(0.,2.57218162001389E-5,4.21568322567862E-5,6.45873314617047E-5,
7.58025810641639E-5,8.14102058653935E-5,8.28121120657009E-5,8.70178306666231E-5,
0.00011608195565799,0.000130526745999935,0.000162394111022053,0.000174035661333246,
0.000213138396956027,0.000256116935429245,0.000302406662848675,0.000348071322666491),
 .UNSPECIFIED.);
#5130=B_SPLINE_CURVE_WITH_KNOTS('',3,(#236552,#236553,#236554,#236555,#236556,
#236557,#236558,#236559,#236560,#236561,#236562,#236563,#236564,#236565,
#236566,#236567,#236568,#236569,#236570,#236571,#236572,#236573,#236574,
#236575,#236576,#236577,#236578,#236579,#236580,#236581,#236582,#236583,
#236584,#236585,#236586,#236587,#236588,#236589,#236590,#236591,#236592,
#236593,#236594,#236595,#236596,#236597,#236598,#236599,#236600,#236601,
#236602,#236603),.UNSPECIFIED.,.F.,.F.,(4,3,3,3,3,3,3,3,3,3,3,3,3,3,3,3,
3,4),(0.,4.2965215217983E-5,8.44519107565792E-5,0.000123669830869106,0.000159788877362988,
0.000170558847912624,0.000181218775907164,0.000181960046452389,0.000214460062643136,
0.000244755726196858,0.000255838271868946,0.000258503253867581,0.000261084955178759,
0.000289370476648369,0.000301101325502013,0.00032110951066364,0.000331113603244454,
0.000341117695825268),.UNSPECIFIED.);
#5131=B_SPLINE_CURVE_WITH_KNOTS('',3,(#236605,#236606,#236607,#236608,#236609,
#236610,#236611,#236612,#236613,#236614,#236615,#236616,#236617,#236618,
#236619,#236620,#236621,#236622,#236623,#236624,#236625,#236626,#236627,
#236628,#236629,#236630,#236631,#236632,#236633,#236634,#236635,#236636,
#236637,#236638,#236639,#236640,#236641,#236642,#236643,#236644,#236645,
#236646,#236647,#236648,#236649,#236650,#236651,#236652,#236653,#236654,
#236655,#236656),.UNSPECIFIED.,.F.,.F.,(4,3,3,3,3,3,3,3,3,3,3,3,3,3,3,3,
3,4),(2.60208521396521E-18,4.30706237866639E-5,8.47417087690563E-5,0.000124159989204738,
0.000160467076288479,0.000170998382116689,0.000182414994733784,0.000213747977645866,
0.000242415955903435,0.000256497573175042,0.000259169422895616,0.000261757777312422,
0.000289965130402706,0.000301877270772909,0.000321937017503152,0.000326951954185713,
0.000334474359209554,0.000341996764233396),.UNSPECIFIED.);
#5132=B_SPLINE_CURVE_WITH_KNOTS('',3,(#236657,#236658,#236659,#236660,#236661,
#236662,#236663,#236664,#236665,#236666,#236667,#236668,#236669,#236670,
#236671,#236672,#236673,#236674,#236675,#236676,#236677,#236678,#236679,
#236680,#236681,#236682,#236683,#236684,#236685,#236686,#236687,#236688,
#236689,#236690,#236691,#236692,#236693,#236694,#236695,#236696,#236697,
#236698,#236699,#236700,#236701,#236702,#236703,#236704,#236705,#236706,
#236707,#236708),.UNSPECIFIED.,.F.,.F.,(4,3,3,3,3,3,3,3,3,3,3,3,3,3,3,3,
3,4),(0.,2.58457451681371E-5,4.25394446196679E-5,6.46659869687498E-5,7.57292581432907E-5,
8.12608937305612E-5,8.26438026273788E-5,8.67925293178317E-5,0.000116015624426802,
0.000130188793976748,0.000151886926306205,0.000161963651211261,0.000162735992470934,
0.000173585058635663,0.000212487880461001,0.000255238173511442,0.000301397761145844,
0.000347170117271343),.UNSPECIFIED.);
#5133=B_SPLINE_CURVE_WITH_KNOTS('',3,(#236710,#236711,#236712,#236713,#236714,
#236715,#236716,#236717,#236718,#236719,#236720,#236721,#236722,#236723,
#236724,#236725,#236726,#236727,#236728,#236729,#236730,#236731,#236732,
#236733,#236734,#236735,#236736,#236737,#236738,#236739,#236740,#236741,
#236742,#236743,#236744,#236745,#236746,#236747,#236748,#236749,#236750,
#236751,#236752,#236753,#236754,#236755),.UNSPECIFIED.,.F.,.F.,(4,3,3,3,
3,3,3,3,3,3,3,3,3,3,3,4),(0.,2.57218161995437E-5,4.21568322568779E-5,6.45873314617477E-5,
7.58025810641826E-5,8.14102058654001E-5,8.28121120657045E-5,8.70178306666175E-5,
0.000116081955658804,0.000130526745999926,0.000162394111022033,0.000174035661333235,
0.000213138396959203,0.000256116935435482,0.00030240666285809,0.00034807132266647),
 .UNSPECIFIED.);
#5134=B_SPLINE_CURVE_WITH_KNOTS('',3,(#236756,#236757,#236758,#236759,#236760,
#236761,#236762,#236763,#236764,#236765,#236766,#236767,#236768,#236769,
#236770,#236771,#236772,#236773,#236774,#236775,#236776,#236777,#236778,
#236779,#236780,#236781,#236782,#236783,#236784,#236785,#236786,#236787,
#236788,#236789,#236790,#236791,#236792,#236793,#236794,#236795,#236796,
#236797,#236798,#236799,#236800,#236801,#236802,#236803,#236804,#236805,
#236806,#236807),.UNSPECIFIED.,.F.,.F.,(4,3,3,3,3,3,3,3,3,3,3,3,3,3,3,3,
3,4),(0.,4.29652152188126E-5,8.44519107580872E-5,0.000123669830871332,0.000159788877365956,
0.000170558847912625,0.000181218775907165,0.000181960046452407,0.000214460062643281,
0.000244755726197407,0.000255838271868945,0.00025850325386758,0.000261084955178758,
0.000289370476647596,0.000301101325502011,0.000321109510663638,0.000331113603244452,
0.000341117695825265),.UNSPECIFIED.);
#5135=B_SPLINE_CURVE_WITH_KNOTS('',3,(#236809,#236810,#236811,#236812,#236813,
#236814,#236815,#236816,#236817,#236818,#236819,#236820,#236821,#236822,
#236823,#236824,#236825,#236826,#236827,#236828,#236829,#236830,#236831,
#236832,#236833,#236834,#236835,#236836,#236837,#236838,#236839,#236840,
#236841,#236842,#236843,#236844,#236845,#236846,#236847,#236848,#236849,
#236850,#236851,#236852,#236853,#236854,#236855,#236856,#236857,#236858,
#236859,#236860),.UNSPECIFIED.,.F.,.F.,(4,3,3,3,3,3,3,3,3,3,3,3,3,3,3,3,
3,4),(2.16840434497101E-18,4.30706237861116E-5,8.47417087683157E-5,0.000124159989204117,
0.000160467076288115,0.000170998382116709,0.000182414994733807,0.00021374797764588,
0.000242415955902621,0.000256497573175051,0.000259169422895624,0.00026175777731243,
0.000289965130403717,0.000301877270772911,0.000321937017503152,0.000326951954185712,
0.000334474359209553,0.000341996764233393),.UNSPECIFIED.);
#5136=B_SPLINE_CURVE_WITH_KNOTS('',3,(#236861,#236862,#236863,#236864,#236865,
#236866,#236867,#236868,#236869,#236870,#236871,#236872,#236873,#236874,
#236875,#236876,#236877,#236878,#236879,#236880,#236881,#236882,#236883,
#236884,#236885,#236886,#236887,#236888,#236889,#236890,#236891,#236892,
#236893,#236894,#236895,#236896,#236897,#236898,#236899,#236900,#236901,
#236902,#236903,#236904,#236905,#236906,#236907,#236908,#236909,#236910,
#236911,#236912),.UNSPECIFIED.,.F.,.F.,(4,3,3,3,3,3,3,3,3,3,3,3,3,3,3,3,
3,4),(0.,2.58457451676982E-5,4.2539444619647E-5,6.46659869687423E-5,7.57292581432899E-5,
8.12608937305638E-5,8.26438026273822E-5,8.67925293178376E-5,0.000116015624426779,
0.000130188793976756,0.000151886926306216,0.000161963651211259,0.000162735992470945,
0.000173585058635675,0.000212487880458101,0.000255238173504257,0.000301397761131382,
0.000347170117271351),.UNSPECIFIED.);
#5137=B_SPLINE_CURVE_WITH_KNOTS('',3,(#236914,#236915,#236916,#236917,#236918,
#236919,#236920,#236921,#236922,#236923,#236924,#236925,#236926,#236927,
#236928,#236929,#236930,#236931,#236932,#236933,#236934,#236935,#236936,
#236937,#236938,#236939,#236940,#236941,#236942,#236943,#236944,#236945,
#236946,#236947,#236948,#236949,#236950,#236951,#236952,#236953,#236954,
#236955,#236956,#236957,#236958,#236959),.UNSPECIFIED.,.F.,.F.,(4,3,3,3,
3,3,3,3,3,3,3,3,3,3,3,4),(0.,2.57218161988846E-5,4.21568322567072E-5,6.45873314616639E-5,
7.58025810641423E-5,8.14102058653814E-5,8.28121120656912E-5,8.70178306666206E-5,
0.000116081955658271,0.000130526745999931,0.000162394111022053,0.000174035661333241,
0.000213138396958831,0.000256116935434894,0.000302406662857592,0.000348071322666483),
 .UNSPECIFIED.);
#5138=B_SPLINE_CURVE_WITH_KNOTS('',3,(#236960,#236961,#236962,#236963,#236964,
#236965,#236966,#236967,#236968,#236969,#236970,#236971,#236972,#236973,
#236974,#236975,#236976,#236977,#236978,#236979,#236980,#236981,#236982,
#236983,#236984,#236985,#236986,#236987,#236988,#236989,#236990,#236991,
#236992,#236993,#236994,#236995,#236996,#236997,#236998,#236999,#237000,
#237001,#237002,#237003,#237004,#237005,#237006,#237007,#237008,#237009,
#237010,#237011),.UNSPECIFIED.,.F.,.F.,(4,3,3,3,3,3,3,3,3,3,3,3,3,3,3,3,
3,4),(1.30104260698261E-18,4.29652152160316E-5,8.44519107531626E-5,0.000123669830864362,
0.000159788877356911,0.000170558847912634,0.000181218775907174,0.000181960046452401,
0.000214460062643762,0.000244755726199148,0.000255838271868951,0.000258503253867586,
0.000261084955178764,0.00028937047664804,0.000301101325502016,0.000321109510663642,
0.000331113603244455,0.000341117695825268),.UNSPECIFIED.);
#5139=B_SPLINE_CURVE_WITH_KNOTS('',3,(#237013,#237014,#237015,#237016,#237017,
#237018,#237019,#237020,#237021,#237022,#237023,#237024,#237025,#237026,
#237027,#237028,#237029,#237030,#237031,#237032,#237033,#237034,#237035,
#237036,#237037,#237038,#237039,#237040,#237041,#237042,#237043,#237044,
#237045,#237046,#237047,#237048,#237049,#237050,#237051,#237052,#237053,
#237054,#237055,#237056,#237057,#237058,#237059,#237060,#237061,#237062,
#237063,#237064),.UNSPECIFIED.,.F.,.F.,(4,3,3,3,3,3,3,3,3,3,3,3,3,3,3,3,
3,4),(4.61009087360184E-18,4.3070623786273E-5,8.47417087683938E-5,0.000124159989203818,
0.000160467076287337,0.000170998382116699,0.000182414994733776,0.000213747977645872,
0.000242415955903083,0.000256497573175046,0.000259169422895619,0.000261757777312424,
0.000289965130403635,0.000301877270772909,0.000321937017503151,0.000326951954185711,
0.000334474359209552,0.000341996764233393),.UNSPECIFIED.);
#5140=B_SPLINE_CURVE_WITH_KNOTS('',3,(#237065,#237066,#237067,#237068,#237069,
#237070,#237071,#237072,#237073,#237074,#237075,#237076,#237077,#237078,
#237079,#237080,#237081,#237082,#237083,#237084,#237085,#237086,#237087,
#237088,#237089,#237090,#237091,#237092,#237093,#237094,#237095,#237096,
#237097,#237098,#237099,#237100,#237101,#237102,#237103,#237104,#237105,
#237106,#237107,#237108,#237109,#237110,#237111,#237112,#237113,#237114,
#237115,#237116),.UNSPECIFIED.,.F.,.F.,(4,3,3,3,3,3,3,3,3,3,3,3,3,3,3,3,
3,4),(0.,2.5845745168412E-5,4.25394446195606E-5,6.46659869687013E-5,7.57292581432716E-5,
8.12608937305567E-5,8.2643802627378E-5,8.67925293178419E-5,0.000116015624427532,
0.000130188793976763,0.000151886926306223,0.000161963651211281,0.000162735992470954,
0.000173585058635684,0.00021248788046143,0.000255238173513324,0.000301397761151222,
0.000347170117271353),.UNSPECIFIED.);
#5141=B_SPLINE_CURVE_WITH_KNOTS('',3,(#237118,#237119,#237120,#237121,#237122,
#237123,#237124,#237125,#237126,#237127,#237128,#237129,#237130,#237131,
#237132,#237133,#237134,#237135,#237136,#237137,#237138,#237139,#237140,
#237141,#237142,#237143,#237144,#237145,#237146,#237147,#237148,#237149,
#237150,#237151,#237152,#237153,#237154,#237155,#237156,#237157,#237158,
#237159,#237160,#237161,#237162,#237163),.UNSPECIFIED.,.F.,.F.,(4,3,3,3,
3,3,3,3,3,3,3,3,3,3,3,4),(3.46944695195361E-18,2.57218161985864E-5,4.21568322567459E-5,
6.45873314616802E-5,7.58025810641474E-5,8.14102058653809E-5,8.28121120656893E-5,
8.70178306666145E-5,0.000116081955657513,0.00013052674599992,0.000162394111022048,
0.000174035661333226,0.000213138396957984,0.000256116935433399,0.000302406662855914,
0.000348071322666466),.UNSPECIFIED.);
#5142=B_SPLINE_CURVE_WITH_KNOTS('',3,(#237164,#237165,#237166,#237167,#237168,
#237169,#237170,#237171,#237172,#237173,#237174,#237175,#237176,#237177,
#237178,#237179,#237180,#237181,#237182,#237183,#237184,#237185,#237186,
#237187,#237188,#237189,#237190,#237191,#237192,#237193,#237194,#237195,
#237196,#237197,#237198,#237199,#237200,#237201,#237202,#237203,#237204,
#237205,#237206,#237207,#237208,#237209,#237210,#237211,#237212,#237213,
#237214,#237215),.UNSPECIFIED.,.F.,.F.,(4,3,3,3,3,3,3,3,3,3,3,3,3,3,3,3,
3,4),(8.67361737988404E-19,4.29652152182944E-5,8.44519107569389E-5,0.000123669830869201,
0.000159788877362635,0.000170558847912625,0.000181218775907165,0.0001819600464524,
0.000214460062643611,0.000244755726198789,0.000255838271868938,0.000258503253867573,
0.00026108495517875,0.000289370476648206,0.000301101325502001,0.000321109510663626,
0.000331113603244438,0.000341117695825251),.UNSPECIFIED.);
#5143=B_SPLINE_CURVE_WITH_KNOTS('',3,(#237217,#237218,#237219,#237220,#237221,
#237222,#237223,#237224,#237225,#237226,#237227,#237228,#237229,#237230,
#237231,#237232,#237233,#237234,#237235,#237236,#237237,#237238,#237239,
#237240,#237241,#237242,#237243,#237244,#237245,#237246,#237247,#237248,
#237249,#237250,#237251,#237252,#237253,#237254,#237255,#237256,#237257,
#237258,#237259,#237260,#237261,#237262,#237263,#237264,#237265,#237266,
#237267,#237268),.UNSPECIFIED.,.F.,.F.,(4,3,3,3,3,3,3,3,3,3,3,3,3,3,3,3,
3,4),(2.16840434497101E-18,4.30706237872889E-5,8.47417087702185E-5,0.000124159989206578,
0.000160467076291047,0.000170998382116701,0.00018241499473378,0.000213747977645874,
0.000242415955903897,0.000256497573175046,0.00025916942289562,0.000261757777312425,
0.00028996513040244,0.000301877270772909,0.00032193701750315,0.000326951954185711,
0.000334474359209551,0.000341996764233392),.UNSPECIFIED.);
#5144=B_SPLINE_CURVE_WITH_KNOTS('',3,(#237269,#237270,#237271,#237272,#237273,
#237274,#237275,#237276,#237277,#237278,#237279,#237280,#237281,#237282,
#237283,#237284,#237285,#237286,#237287,#237288,#237289,#237290,#237291,
#237292,#237293,#237294,#237295,#237296,#237297,#237298,#237299,#237300,
#237301,#237302,#237303,#237304,#237305,#237306,#237307,#237308,#237309,
#237310,#237311,#237312,#237313,#237314,#237315,#237316,#237317,#237318,
#237319,#237320),.UNSPECIFIED.,.F.,.F.,(4,3,3,3,3,3,3,3,3,3,3,3,3,3,3,3,
3,4),(3.46944695195361E-18,2.58457451676127E-5,4.25394446194762E-5,6.46659869686576E-5,
7.57292581432484E-5,8.12608937305437E-5,8.26438026273676E-5,8.67925293178391E-5,
0.000116015624427052,0.000130188793976757,0.000151886926306216,0.000161963651211258,
0.000162735992470945,0.000173585058635675,0.000212487880458538,0.000255238173506317,
0.000301397761137294,0.000347170117271365),.UNSPECIFIED.);
#5145=B_SPLINE_CURVE_WITH_KNOTS('',3,(#237322,#237323,#237324,#237325,#237326,
#237327,#237328,#237329,#237330,#237331,#237332,#237333,#237334,#237335,
#237336,#237337,#237338,#237339,#237340,#237341,#237342,#237343,#237344,
#237345,#237346,#237347,#237348,#237349,#237350,#237351,#237352,#237353,
#237354,#237355,#237356,#237357,#237358,#237359,#237360,#237361,#237362,
#237363,#237364,#237365,#237366,#237367),.UNSPECIFIED.,.F.,.F.,(4,3,3,3,
3,3,3,3,3,3,3,3,3,3,3,4),(3.46944695195361E-18,2.5721816201202E-5,4.21568322569165E-5,
6.45873314617695E-5,7.5802581064196E-5,8.14102058654092E-5,8.28121120657125E-5,
8.70178306666225E-5,0.000116081955659048,0.000130526745999932,0.000162394111022063,
0.000174035661333241,0.000213138396958407,0.000256116935434203,0.000302406662857052,
0.000348071322666463),.UNSPECIFIED.);
#5146=B_SPLINE_CURVE_WITH_KNOTS('',3,(#237368,#237369,#237370,#237371,#237372,
#237373,#237374,#237375,#237376,#237377,#237378,#237379,#237380,#237381,
#237382,#237383,#237384,#237385,#237386,#237387,#237388,#237389,#237390,
#237391,#237392,#237393,#237394,#237395,#237396,#237397,#237398,#237399,
#237400,#237401,#237402,#237403,#237404,#237405,#237406,#237407,#237408,
#237409,#237410,#237411,#237412,#237413,#237414,#237415,#237416,#237417,
#237418,#237419),.UNSPECIFIED.,.F.,.F.,(4,3,3,3,3,3,3,3,3,3,3,3,3,3,3,3,
3,4),(0.,4.29652152166832E-5,8.44519107542356E-5,0.000123669830865694,0.000159788877358465,
0.000170558847912624,0.000181218775907163,0.0001819600464524,0.000214460062643199,
0.000244755726197238,0.000255838271868937,0.000258503253867572,0.00026108495517875,
0.000289370476648487,0.000301101325502,0.000321109510663625,0.000331113603244438,
0.00034111769582525),.UNSPECIFIED.);
#5147=B_SPLINE_CURVE_WITH_KNOTS('',3,(#237421,#237422,#237423,#237424,#237425,
#237426,#237427,#237428,#237429,#237430,#237431,#237432,#237433,#237434,
#237435,#237436,#237437,#237438,#237439,#237440,#237441,#237442,#237443,
#237444,#237445,#237446,#237447,#237448,#237449,#237450,#237451,#237452,
#237453,#237454,#237455,#237456,#237457,#237458,#237459,#237460,#237461,
#237462,#237463,#237464,#237465,#237466,#237467,#237468,#237469,#237470,
#237471,#237472),.UNSPECIFIED.,.F.,.F.,(4,3,3,3,3,3,3,3,3,3,3,3,3,3,3,3,
3,4),(1.0702344114451E-17,4.30706237862214E-5,8.47417087682975E-5,0.000124159989203744,
0.000160467076287253,0.000170998382116703,0.000182414994733785,0.000213747977645876,
0.000242415955902651,0.000256497573175048,0.000259169422895622,0.000261757777312427,
0.000289965130403741,0.00030187727077291,0.000321937017503152,0.000326951954185712,
0.000334474359209553,0.000341996764233393),.UNSPECIFIED.);
#5148=B_SPLINE_CURVE_WITH_KNOTS('',3,(#237473,#237474,#237475,#237476,#237477,
#237478,#237479,#237480,#237481,#237482,#237483,#237484,#237485,#237486,
#237487,#237488,#237489,#237490,#237491,#237492,#237493,#237494,#237495,
#237496,#237497,#237498,#237499,#237500,#237501,#237502,#237503,#237504,
#237505,#237506,#237507,#237508,#237509,#237510,#237511,#237512,#237513,
#237514,#237515,#237516,#237517,#237518,#237519,#237520,#237521,#237522,
#237523,#237524),.UNSPECIFIED.,.F.,.F.,(4,3,3,3,3,3,3,3,3,3,3,3,3,3,3,3,
3,4),(1.73472347597681E-18,2.58457451676447E-5,4.25394446196667E-5,6.46659869687532E-5,
7.57292581432965E-5,8.12608937305681E-5,8.2643802627386E-5,8.67925293178398E-5,
0.000116015624427285,0.000130188793976759,0.000151886926306218,0.00016196365121126,
0.000162735992470948,0.000173585058635678,0.000212487880458775,0.000255238173506902,
0.000301397761138638,0.000347170117271369),.UNSPECIFIED.);
#5149=B_SPLINE_CURVE_WITH_KNOTS('',3,(#237526,#237527,#237528,#237529,#237530,
#237531,#237532,#237533,#237534,#237535,#237536,#237537,#237538,#237539,
#237540,#237541,#237542,#237543,#237544,#237545,#237546,#237547,#237548,
#237549,#237550,#237551,#237552,#237553,#237554,#237555,#237556,#237557,
#237558,#237559,#237560,#237561,#237562,#237563,#237564,#237565,#237566,
#237567,#237568,#237569,#237570,#237571),.UNSPECIFIED.,.F.,.F.,(4,3,3,3,
3,3,3,3,3,3,3,3,3,3,3,4),(0.,2.57218161997054E-5,4.2156832256664E-5,6.45873314616409E-5,
7.58025810641293E-5,8.14102058653735E-5,8.28121120656845E-5,8.70178306666177E-5,
0.00011608195565801,0.000130526745999927,0.000162394111022051,0.000174035661333235,
0.000213138396956663,0.000256116935430629,0.000302406662851181,0.000348071322666486),
 .UNSPECIFIED.);
#5150=B_SPLINE_CURVE_WITH_KNOTS('',3,(#237572,#237573,#237574,#237575,#237576,
#237577,#237578,#237579,#237580,#237581,#237582,#237583,#237584,#237585,
#237586,#237587,#237588,#237589,#237590,#237591,#237592,#237593,#237594,
#237595,#237596,#237597,#237598,#237599,#237600,#237601,#237602,#237603,
#237604,#237605,#237606,#237607,#237608,#237609,#237610,#237611,#237612,
#237613,#237614,#237615,#237616,#237617,#237618,#237619,#237620,#237621,
#237622,#237623),.UNSPECIFIED.,.F.,.F.,(4,3,3,3,3,3,3,3,3,3,3,3,3,3,3,3,
3,4),(4.33680868994202E-19,4.29652152129658E-5,8.44519107482501E-5,0.000123669830858316,
0.000159788877350148,0.000170558847912625,0.000181218775907164,0.000181960046452394,
0.000214460062643421,0.000244755726197445,0.000255838271868942,0.000258503253867577,
0.000261084955178755,0.000289370476647996,0.000301101325502007,0.000321109510663633,
0.000331113603244447,0.00034111769582526),.UNSPECIFIED.);
#5151=B_SPLINE_CURVE_WITH_KNOTS('',3,(#237625,#237626,#237627,#237628,#237629,
#237630,#237631,#237632,#237633,#237634,#237635,#237636,#237637,#237638,
#237639,#237640,#237641,#237642,#237643,#237644,#237645,#237646,#237647,
#237648,#237649,#237650,#237651,#237652,#237653,#237654,#237655,#237656,
#237657,#237658,#237659,#237660,#237661,#237662,#237663,#237664,#237665,
#237666,#237667,#237668,#237669,#237670,#237671,#237672,#237673,#237674,
#237675,#237676),.UNSPECIFIED.,.F.,.F.,(4,3,3,3,3,3,3,3,3,3,3,3,3,3,3,3,
3,4),(9.66826306931024E-18,4.30706237866843E-5,8.4741708768988E-5,0.000124159989204507,
0.000160467076288014,0.000170998382116706,0.000182414994733798,0.000213747977645878,
0.000242415955902607,0.000256497573175049,0.000259169422895622,0.000261757777312428,
0.000289965130403992,0.00030187727077291,0.000321937017503151,0.000326951954185711,
0.000334474359209552,0.000341996764233392),.UNSPECIFIED.);
#5152=B_SPLINE_CURVE_WITH_KNOTS('',3,(#237677,#237678,#237679,#237680,#237681,
#237682,#237683,#237684,#237685,#237686,#237687,#237688,#237689,#237690,
#237691,#237692,#237693,#237694,#237695,#237696,#237697,#237698,#237699,
#237700,#237701,#237702,#237703,#237704,#237705,#237706,#237707,#237708,
#237709,#237710,#237711,#237712,#237713,#237714,#237715,#237716,#237717,
#237718,#237719,#237720,#237721,#237722,#237723,#237724,#237725,#237726,
#237727,#237728),.UNSPECIFIED.,.F.,.F.,(4,3,3,3,3,3,3,3,3,3,3,3,3,3,3,3,
3,4),(0.,2.58457451676031E-5,4.25394446196135E-5,6.46659869687281E-5,7.57292581432855E-5,
8.12608937305641E-5,8.26438026273838E-5,8.67925293178428E-5,0.000116015624427197,
0.000130188793976764,0.000151886926306225,0.000161963651211278,0.000162735992470955,
0.000173585058635686,0.000212487880462397,0.000255238173513979,0.000301397761149119,
0.00034717011727137),.UNSPECIFIED.);
#5153=B_SPLINE_CURVE_WITH_KNOTS('',3,(#237730,#237731,#237732,#237733,#237734,
#237735,#237736,#237737,#237738,#237739,#237740,#237741,#237742,#237743,
#237744,#237745,#237746,#237747,#237748,#237749,#237750,#237751,#237752,
#237753,#237754,#237755,#237756,#237757,#237758,#237759,#237760,#237761,
#237762,#237763,#237764,#237765,#237766,#237767,#237768,#237769,#237770,
#237771,#237772,#237773,#237774,#237775),.UNSPECIFIED.,.F.,.F.,(4,3,3,3,
3,3,3,3,3,3,3,3,3,3,3,4),(8.67361737988404E-19,2.57218161993305E-5,4.21568322567911E-5,
6.45873314617076E-5,7.58025810641659E-5,8.1410205865395E-5,8.28121120657023E-5,
8.70178306666241E-5,0.000116081955658071,0.000130526745999936,0.00016239411102206,
0.000174035661333247,0.000213138396957183,0.000256116935431462,0.000302406662851793,
0.000348071322666493),.UNSPECIFIED.);
#5154=B_SPLINE_CURVE_WITH_KNOTS('',3,(#237776,#237777,#237778,#237779,#237780,
#237781,#237782,#237783,#237784,#237785,#237786,#237787,#237788,#237789,
#237790,#237791,#237792,#237793,#237794,#237795,#237796,#237797,#237798,
#237799,#237800,#237801,#237802,#237803,#237804,#237805,#237806,#237807,
#237808,#237809,#237810,#237811,#237812,#237813,#237814,#237815,#237816,
#237817,#237818,#237819,#237820,#237821,#237822,#237823,#237824,#237825,
#237826,#237827),.UNSPECIFIED.,.F.,.F.,(4,3,3,3,3,3,3,3,3,3,3,3,3,3,3,3,
3,4),(0.,4.29652152133897E-5,8.44519107489504E-5,0.00012366983085924,0.000159788877351311,
0.000170558847912625,0.000181218775907164,0.000181960046452397,0.000214460062643666,
0.000244755726198589,0.000255838271868937,0.000258503253867572,0.000261084955178749,
0.000289370476647751,0.000301101325502,0.000321109510663625,0.000331113603244437,
0.00034111769582525),.UNSPECIFIED.);
#5155=B_SPLINE_CURVE_WITH_KNOTS('',3,(#237829,#237830,#237831,#237832,#237833,
#237834,#237835,#237836,#237837,#237838,#237839,#237840,#237841,#237842,
#237843,#237844,#237845,#237846,#237847,#237848,#237849,#237850,#237851,
#237852,#237853,#237854,#237855,#237856,#237857,#237858,#237859,#237860,
#237861,#237862,#237863,#237864,#237865,#237866,#237867,#237868,#237869,
#237870,#237871,#237872,#237873,#237874,#237875,#237876,#237877,#237878,
#237879,#237880),.UNSPECIFIED.,.F.,.F.,(4,3,3,3,3,3,3,3,3,3,3,3,3,3,3,3,
3,4),(3.09377807083354E-18,4.30706237871686E-5,8.47417087700116E-5,0.000124159989206186,
0.000160467076290512,0.000170998382116679,0.000182414994733741,0.000213747977645855,
0.000242415955903015,0.00025649757317503,0.000259169422895604,0.000261757777312409,
0.000289965130403648,0.000301877270772895,0.000321937017503138,0.000326951954185699,
0.00033447435920954,0.000341996764233381),.UNSPECIFIED.);
#5156=B_SPLINE_CURVE_WITH_KNOTS('',3,(#237881,#237882,#237883,#237884,#237885,
#237886,#237887,#237888,#237889,#237890,#237891,#237892,#237893,#237894,
#237895,#237896,#237897,#237898,#237899,#237900,#237901,#237902,#237903,
#237904,#237905,#237906,#237907,#237908,#237909,#237910,#237911,#237912,
#237913,#237914,#237915,#237916,#237917,#237918,#237919,#237920,#237921,
#237922,#237923,#237924,#237925,#237926,#237927,#237928,#237929,#237930,
#237931,#237932),.UNSPECIFIED.,.F.,.F.,(4,3,3,3,3,3,3,3,3,3,3,3,3,3,3,3,
3,4),(0.,2.58457451678914E-5,4.2539444619683E-5,6.46659869687625E-5,7.57292581433022E-5,
8.12608937305721E-5,8.26438026273895E-5,8.67925293178419E-5,0.000116015624427083,
0.000130188793976763,0.000151886926306223,0.000161963651211268,0.000162735992470954,
0.000173585058635684,0.000212487880460161,0.000255238173510438,0.000301397761145908,
0.000347170117271354),.UNSPECIFIED.);
#5157=B_SPLINE_CURVE_WITH_KNOTS('',3,(#237934,#237935,#237936,#237937,#237938,
#237939,#237940,#237941,#237942,#237943,#237944,#237945,#237946,#237947,
#237948,#237949,#237950,#237951,#237952,#237953,#237954,#237955,#237956,
#237957,#237958,#237959,#237960,#237961,#237962,#237963,#237964,#237965,
#237966,#237967,#237968,#237969,#237970,#237971,#237972,#237973,#237974,
#237975,#237976,#237977,#237978,#237979),.UNSPECIFIED.,.F.,.F.,(4,3,3,3,
3,3,3,3,3,3,3,3,3,3,3,4),(2.74438674910393E-19,2.5721816198343E-5,4.21568322569397E-5,
6.45873314617789E-5,7.58025810641984E-5,8.14102058654082E-5,8.28121120657107E-5,
8.7017830666618E-5,0.000116081955658225,0.000130526745999927,0.00016239411102205,
0.000174035661333236,0.000213138396959223,0.000256116935435911,0.000302406662859976,
0.000348071322666472),.UNSPECIFIED.);
#5158=B_SPLINE_CURVE_WITH_KNOTS('',3,(#237980,#237981,#237982,#237983,#237984,
#237985,#237986,#237987,#237988,#237989,#237990,#237991,#237992,#237993,
#237994,#237995,#237996,#237997,#237998,#237999,#238000,#238001,#238002,
#238003,#238004,#238005,#238006,#238007,#238008,#238009,#238010,#238011,
#238012,#238013,#238014,#238015,#238016,#238017,#238018,#238019,#238020,
#238021,#238022,#238023,#238024,#238025,#238026,#238027,#238028,#238029,
#238030,#238031),.UNSPECIFIED.,.F.,.F.,(4,3,3,3,3,3,3,3,3,3,3,3,3,3,3,3,
3,4),(0.,4.29652152174176E-5,8.445191075561E-5,0.000123669830867732,0.000159788877361313,
0.000170558847912633,0.000181218775907173,0.000181960046452402,0.000214460062643273,
0.000244755726197394,0.00025583827186895,0.000258503253867585,0.000261084955178762,
0.000289370476648092,0.000301101325502014,0.00032110951066364,0.000331113603244453,
0.000341117695825266),.UNSPECIFIED.);
#5159=B_SPLINE_CURVE_WITH_KNOTS('',3,(#238033,#238034,#238035,#238036,#238037,
#238038,#238039,#238040,#238041,#238042,#238043,#238044,#238045,#238046,
#238047,#238048,#238049,#238050,#238051,#238052,#238053,#238054,#238055,
#238056,#238057,#238058,#238059,#238060,#238061,#238062,#238063,#238064,
#238065,#238066,#238067,#238068,#238069,#238070,#238071,#238072,#238073,
#238074,#238075,#238076,#238077,#238078,#238079,#238080,#238081,#238082,
#238083,#238084),.UNSPECIFIED.,.F.,.F.,(4,3,3,3,3,3,3,3,3,3,3,3,3,3,3,3,
3,4),(4.33680868994202E-19,4.30706237870913E-5,8.47417087699565E-5,0.000124159989206289,
0.000160467076290841,0.000170998382116694,0.000182414994733777,0.000213747977645867,
0.000242415955902843,0.00025649757317504,0.000259169422895614,0.000261757777312419,
0.000289965130403804,0.000301877270772903,0.000321937017503145,0.000326951954185706,
0.000334474359209546,0.000341996764233387),.UNSPECIFIED.);
#5160=B_SPLINE_CURVE_WITH_KNOTS('',3,(#238085,#238086,#238087,#238088,#238089,
#238090,#238091,#238092,#238093,#238094,#238095,#238096,#238097,#238098,
#238099,#238100,#238101,#238102,#238103,#238104,#238105,#238106,#238107,
#238108,#238109,#238110,#238111,#238112,#238113,#238114,#238115,#238116,
#238117,#238118,#238119,#238120,#238121,#238122,#238123,#238124,#238125,
#238126,#238127,#238128,#238129,#238130,#238131,#238132,#238133,#238134,
#238135,#238136),.UNSPECIFIED.,.F.,.F.,(4,3,3,3,3,3,3,3,3,3,3,3,3,3,3,3,
3,4),(0.,2.58457451666468E-5,4.25394446196103E-5,6.46659869687272E-5,7.57292581432856E-5,
8.12608937305648E-5,8.26438026273846E-5,8.6792529317844E-5,0.000116015624426662,
0.000130188793976766,0.000151886926306227,0.000161963651211283,0.000162735992470958,
0.000173585058635688,0.000212487880463352,0.000255238173516254,0.000301397761153875,
0.000347170117271378),.UNSPECIFIED.);
#5161=B_SPLINE_CURVE_WITH_KNOTS('',3,(#238138,#238139,#238140,#238141,#238142,
#238143,#238144,#238145,#238146,#238147,#238148,#238149,#238150,#238151,
#238152,#238153,#238154,#238155,#238156,#238157,#238158,#238159,#238160,
#238161,#238162,#238163,#238164,#238165,#238166,#238167,#238168,#238169,
#238170,#238171,#238172,#238173,#238174,#238175,#238176,#238177,#238178,
#238179,#238180,#238181,#238182,#238183),.UNSPECIFIED.,.F.,.F.,(4,3,3,3,
3,3,3,3,3,3,3,3,3,3,3,4),(8.67361737988404E-19,2.57218161983997E-5,4.21568322567976E-5,
6.45873314617104E-5,7.58025810641669E-5,8.14102058653951E-5,8.28121120657021E-5,
8.70178306666233E-5,0.000116081955658178,0.000130526745999931,0.000162394111022045,
0.000174035661333238,0.0002131383969601,0.000256116935437471,0.000302406662861761,
0.000348071322666481),.UNSPECIFIED.);
#5162=B_SPLINE_CURVE_WITH_KNOTS('',3,(#238184,#238185,#238186,#238187,#238188,
#238189,#238190,#238191,#238192,#238193,#238194,#238195,#238196,#238197,
#238198,#238199,#238200,#238201,#238202,#238203,#238204,#238205,#238206,
#238207,#238208,#238209,#238210,#238211,#238212,#238213,#238214,#238215,
#238216,#238217,#238218,#238219,#238220,#238221,#238222,#238223,#238224,
#238225,#238226,#238227,#238228,#238229,#238230,#238231,#238232,#238233,
#238234,#238235),.UNSPECIFIED.,.F.,.F.,(4,3,3,3,3,3,3,3,3,3,3,3,3,3,3,3,
3,4),(0.,4.29652152176474E-5,8.44519107560601E-5,0.00012366983086853,0.000159788877362454,
0.000170558847912624,0.000181218775907163,0.000181960046452395,0.000214460062643399,
0.000244755726197756,0.000255838271868942,0.000258503253867577,0.000261084955178754,
0.000289370476647851,0.000301101325502007,0.000321109510663634,0.000331113603244447,
0.00034111769582526),.UNSPECIFIED.);
#5163=B_SPLINE_CURVE_WITH_KNOTS('',3,(#238237,#238238,#238239,#238240,#238241,
#238242,#238243,#238244,#238245,#238246,#238247,#238248,#238249,#238250,
#238251,#238252,#238253,#238254,#238255,#238256,#238257,#238258,#238259,
#238260,#238261,#238262,#238263,#238264,#238265,#238266,#238267,#238268,
#238269,#238270,#238271,#238272,#238273,#238274,#238275,#238276,#238277,
#238278,#238279,#238280,#238281,#238282,#238283,#238284,#238285,#238286,
#238287,#238288),.UNSPECIFIED.,.F.,.F.,(4,3,3,3,3,3,3,3,3,3,3,3,3,3,3,3,
3,4),(3.03576608295941E-18,4.30706237872062E-5,8.47417087700904E-5,0.000124159989206327,
0.000160467076290739,0.000170998382116701,0.000182414994733785,0.000213747977645875,
0.000242415955903026,0.000256497573175049,0.000259169422895622,0.000261757777312428,
0.000289965130403995,0.000301877270772912,0.000321937017503155,0.000326951954185715,
0.000334474359209556,0.000341996764233397),.UNSPECIFIED.);
#5164=B_SPLINE_CURVE_WITH_KNOTS('',3,(#238289,#238290,#238291,#238292,#238293,
#238294,#238295,#238296,#238297,#238298,#238299,#238300,#238301,#238302,
#238303,#238304,#238305,#238306,#238307,#238308,#238309,#238310,#238311,
#238312,#238313,#238314,#238315,#238316,#238317,#238318,#238319,#238320,
#238321,#238322,#238323,#238324,#238325,#238326,#238327,#238328,#238329,
#238330,#238331,#238332,#238333,#238334,#238335,#238336,#238337,#238338,
#238339,#238340),.UNSPECIFIED.,.F.,.F.,(4,3,3,3,3,3,3,3,3,3,3,3,3,3,3,3,
3,4),(0.,2.58457451677985E-5,4.25394446195654E-5,6.46659869687035E-5,7.57292581432725E-5,
8.1260893730557E-5,8.26438026273782E-5,8.67925293178416E-5,0.000116015624427485,
0.000130188793976762,0.000151886926306223,0.000161963651211287,0.000162735992470953,
0.000173585058635683,0.000212487880460691,0.00025523817351173,0.000301397761148335,
0.000347170117271366),.UNSPECIFIED.);
#5165=B_SPLINE_CURVE_WITH_KNOTS('',3,(#238342,#238343,#238344,#238345,#238346,
#238347,#238348,#238349,#238350,#238351,#238352,#238353,#238354,#238355,
#238356,#238357,#238358,#238359,#238360,#238361,#238362,#238363,#238364,
#238365,#238366,#238367,#238368,#238369,#238370,#238371,#238372,#238373,
#238374,#238375,#238376,#238377,#238378,#238379,#238380,#238381,#238382,
#238383,#238384,#238385,#238386,#238387),.UNSPECIFIED.,.F.,.F.,(4,3,3,3,
3,3,3,3,3,3,3,3,3,3,3,4),(0.,2.57218161992493E-5,4.215683225679E-5,6.45873314617063E-5,
7.58025810641645E-5,8.14102058653936E-5,8.28121120657009E-5,8.70178306666227E-5,
0.000116081955658092,0.000130526745999934,0.000162394111022042,0.000174035661333245,
0.000213138396956871,0.000256116935430989,0.000302406662851721,0.000348071322666493),
 .UNSPECIFIED.);
#5166=B_SPLINE_CURVE_WITH_KNOTS('',3,(#238388,#238389,#238390,#238391,#238392,
#238393,#238394,#238395,#238396,#238397,#238398,#238399,#238400,#238401,
#238402,#238403,#238404,#238405,#238406,#238407,#238408,#238409,#238410,
#238411,#238412,#238413,#238414,#238415,#238416,#238417,#238418,#238419,
#238420,#238421,#238422,#238423,#238424,#238425,#238426,#238427,#238428,
#238429,#238430,#238431,#238432,#238433,#238434,#238435,#238436,#238437,
#238438,#238439),.UNSPECIFIED.,.F.,.F.,(4,3,3,3,3,3,3,3,3,3,3,3,3,3,3,3,
3,4),(3.03576608295941E-18,4.29652152151958E-5,8.44519107520227E-5,0.000123669830863345,
0.000159788877356407,0.000170558847912634,0.000181218775907174,0.000181960046452411,
0.000214460062643647,0.000244755726198505,0.000255838271868951,0.000258503253867586,
0.000261084955178763,0.000289370476647687,0.000301101325502015,0.000321109510663641,
0.000331113603244454,0.000341117695825267),.UNSPECIFIED.);
#5167=B_SPLINE_CURVE_WITH_KNOTS('',3,(#238441,#238442,#238443,#238444,#238445,
#238446,#238447,#238448,#238449,#238450,#238451,#238452,#238453,#238454,
#238455,#238456,#238457,#238458,#238459,#238460,#238461,#238462,#238463,
#238464,#238465,#238466,#238467,#238468,#238469,#238470,#238471,#238472,
#238473,#238474,#238475,#238476,#238477,#238478,#238479,#238480,#238481,
#238482,#238483,#238484,#238485,#238486,#238487,#238488,#238489,#238490,
#238491,#238492),.UNSPECIFIED.,.F.,.F.,(4,3,3,3,3,3,3,3,3,3,3,3,3,3,3,3,
3,4),(4.33680868994202E-19,4.3070623784098E-5,8.4741708764398E-5,0.000124159989198101,
0.000160467076279639,0.000170998382116699,0.000182414994733788,0.00021374797764587,
0.000242415955902635,0.000256497573175042,0.000259169422895615,0.00026175777731242,
0.000289965130405031,0.000301877270772902,0.000321937017503143,0.000326951954185704,
0.000334474359209544,0.000341996764233385),.UNSPECIFIED.);
#5168=B_SPLINE_CURVE_WITH_KNOTS('',3,(#238493,#238494,#238495,#238496,#238497,
#238498,#238499,#238500,#238501,#238502,#238503,#238504,#238505,#238506,
#238507,#238508,#238509,#238510,#238511,#238512,#238513,#238514,#238515,
#238516,#238517,#238518,#238519,#238520,#238521,#238522,#238523,#238524,
#238525,#238526,#238527,#238528,#238529,#238530,#238531,#238532,#238533,
#238534,#238535,#238536,#238537,#238538,#238539,#238540,#238541,#238542,
#238543,#238544),.UNSPECIFIED.,.F.,.F.,(4,3,3,3,3,3,3,3,3,3,3,3,3,3,3,3,
3,4),(3.46944695195361E-18,2.5845745167508E-5,4.25394446194645E-5,6.46659869686533E-5,
7.57292581432477E-5,8.12608937305449E-5,8.26438026273692E-5,8.67925293178421E-5,
0.00011601562442678,0.000130188793976761,0.000151886926306221,0.000161963651211275,
0.000162735992470951,0.000173585058635681,0.000212487880460457,0.000255238173511178,
0.000301397761147439,0.000347170117271366),.UNSPECIFIED.);
#5169=B_SPLINE_CURVE_WITH_KNOTS('',3,(#238546,#238547,#238548,#238549,#238550,
#238551,#238552,#238553,#238554,#238555,#238556,#238557,#238558,#238559,
#238560,#238561,#238562,#238563,#238564,#238565,#238566,#238567,#238568,
#238569,#238570,#238571,#238572,#238573,#238574,#238575,#238576,#238577,
#238578,#238579,#238580,#238581,#238582,#238583,#238584,#238585,#238586,
#238587,#238588,#238589,#238590,#238591),.UNSPECIFIED.,.F.,.F.,(4,3,3,3,
3,3,3,3,3,3,3,3,3,3,3,4),(0.,2.57218161987356E-5,4.21568322568225E-5,6.45873314617223E-5,
7.58025810641722E-5,8.14102058653971E-5,8.28121120657033E-5,8.7017830666622E-5,
0.000116081955657996,0.000130526745999933,0.000162394111022048,0.000174035661333244,
0.000213138396959427,0.000256116935436209,0.000302406662860123,0.000348071322666472),
 .UNSPECIFIED.);
#5170=B_SPLINE_CURVE_WITH_KNOTS('',3,(#238592,#238593,#238594,#238595,#238596,
#238597,#238598,#238599,#238600,#238601,#238602,#238603,#238604,#238605,
#238606,#238607,#238608,#238609,#238610,#238611,#238612,#238613,#238614,
#238615,#238616,#238617,#238618,#238619,#238620,#238621,#238622,#238623,
#238624,#238625,#238626,#238627,#238628,#238629,#238630,#238631,#238632,
#238633,#238634,#238635,#238636,#238637,#238638,#238639,#238640,#238641,
#238642,#238643),.UNSPECIFIED.,.F.,.F.,(4,3,3,3,3,3,3,3,3,3,3,3,3,3,3,3,
3,4),(4.33680868994202E-19,4.29652152166818E-5,8.44519107542978E-5,0.000123669830865928,
0.000159788877358893,0.000170558847912628,0.000181218775907169,0.000181960046452395,
0.000214460062643088,0.000244755726196831,0.00025583827186895,0.000258503253867585,
0.000261084955178763,0.000289370476648246,0.000301101325502018,0.000321109510663645,
0.000331113603244458,0.000341117695825272),.UNSPECIFIED.);
#5171=B_SPLINE_CURVE_WITH_KNOTS('',3,(#238645,#238646,#238647,#238648,#238649,
#238650,#238651,#238652,#238653,#238654,#238655,#238656,#238657,#238658,
#238659,#238660,#238661,#238662,#238663,#238664,#238665,#238666,#238667,
#238668,#238669,#238670,#238671,#238672,#238673,#238674,#238675,#238676,
#238677,#238678,#238679,#238680,#238681,#238682,#238683,#238684,#238685,
#238686,#238687,#238688,#238689,#238690,#238691,#238692,#238693,#238694,
#238695,#238696),.UNSPECIFIED.,.F.,.F.,(4,3,3,3,3,3,3,3,3,3,3,3,3,3,3,3,
3,4),(0.,4.30706237880981E-5,8.47417087717393E-5,0.000124159989208782,0.000160467076294121,
0.000170998382116685,0.000182414994733763,0.000213747977645861,0.000242415955903088,
0.000256497573175037,0.00025916942289561,0.000261757777312416,0.000289965130403175,
0.000301877270772902,0.000321937017503145,0.000326951954185706,0.000334474359209547,
0.000341996764233388),.UNSPECIFIED.);
#5172=B_SPLINE_CURVE_WITH_KNOTS('',3,(#238697,#238698,#238699,#238700,#238701,
#238702,#238703,#238704,#238705,#238706,#238707,#238708,#238709,#238710,
#238711,#238712,#238713,#238714,#238715,#238716,#238717,#238718,#238719,
#238720,#238721,#238722,#238723,#238724,#238725,#238726,#238727,#238728,
#238729,#238730,#238731,#238732,#238733,#238734,#238735,#238736,#238737,
#238738,#238739,#238740,#238741,#238742,#238743,#238744,#238745,#238746,
#238747,#238748),.UNSPECIFIED.,.F.,.F.,(4,3,3,3,3,3,3,3,3,3,3,3,3,3,3,3,
3,4),(0.,2.5845745168441E-5,4.25394446196211E-5,6.46659869687328E-5,7.57292581432887E-5,
8.12608937305666E-5,8.26438026273861E-5,8.67925293178446E-5,0.000116015624426974,
0.000130188793976767,0.000151886926306228,0.000161963651211272,0.000162735992470959,
0.000173585058635689,0.000212487880461697,0.000255238173513341,0.000301397761150061,
0.000347170117271378),.UNSPECIFIED.);
#5173=B_SPLINE_CURVE_WITH_KNOTS('',3,(#238750,#238751,#238752,#238753,#238754,
#238755,#238756,#238757,#238758,#238759,#238760,#238761,#238762,#238763,
#238764,#238765,#238766,#238767,#238768,#238769,#238770,#238771,#238772,
#238773,#238774,#238775,#238776,#238777,#238778,#238779,#238780,#238781,
#238782,#238783,#238784,#238785,#238786,#238787,#238788,#238789,#238790,
#238791,#238792,#238793,#238794,#238795),.UNSPECIFIED.,.F.,.F.,(4,3,3,3,
3,3,3,3,3,3,3,3,3,3,3,4),(0.,2.57218162001823E-5,4.21568322568501E-5,6.45873314617339E-5,
7.58025810641758E-5,8.14102058653967E-5,8.2812112065702E-5,8.70178306666177E-5,
0.000116081955658371,0.000130526745999927,0.000162394111022044,0.000174035661333235,
0.000213138396959927,0.000256116935437149,0.000302406662861384,0.000348071322666479),
 .UNSPECIFIED.);
#5174=B_SPLINE_CURVE_WITH_KNOTS('',3,(#238796,#238797,#238798,#238799,#238800,
#238801,#238802,#238803,#238804,#238805,#238806,#238807,#238808,#238809,
#238810,#238811,#238812,#238813,#238814,#238815,#238816,#238817,#238818,
#238819,#238820,#238821,#238822,#238823,#238824,#238825,#238826,#238827,
#238828,#238829,#238830,#238831,#238832,#238833,#238834,#238835,#238836,
#238837,#238838,#238839,#238840,#238841,#238842,#238843,#238844,#238845,
#238846,#238847),.UNSPECIFIED.,.F.,.F.,(4,3,3,3,3,3,3,3,3,3,3,3,3,3,3,3,
3,4),(8.67361737988404E-19,4.29652152182224E-5,8.44519107567866E-5,0.000123669830869072,
0.000159788877362546,0.000170558847912642,0.000181218775907181,0.000181960046452415,
0.000214460062643632,0.000244755726198693,0.000255838271868955,0.000258503253867589,
0.000261084955178767,0.000289370476647603,0.000301101325502017,0.000321109510663642,
0.000331113603244455,0.000341117695825267),.UNSPECIFIED.);
#5175=B_SPLINE_CURVE_WITH_KNOTS('',3,(#238849,#238850,#238851,#238852,#238853,
#238854,#238855,#238856,#238857,#238858,#238859,#238860,#238861,#238862,
#238863,#238864,#238865,#238866,#238867,#238868,#238869,#238870,#238871,
#238872,#238873,#238874,#238875,#238876,#238877,#238878,#238879,#238880,
#238881,#238882,#238883,#238884,#238885,#238886,#238887,#238888,#238889,
#238890,#238891,#238892,#238893,#238894,#238895,#238896,#238897,#238898,
#238899,#238900),.UNSPECIFIED.,.F.,.F.,(4,3,3,3,3,3,3,3,3,3,3,3,3,3,3,3,
3,4),(0.,4.3070623782646E-5,8.47417087619512E-5,0.000124159989194811,0.00016046707627559,
0.000170998382116695,0.00018241499473379,0.000213747977645869,0.00024241595590369,
0.000256497573175043,0.000259169422895617,0.000261757777312422,0.000289965130404861,
0.000301877270772907,0.000321937017503149,0.000326951954185709,0.00033447435920955,
0.000341996764233391),.UNSPECIFIED.);
#5176=B_SPLINE_CURVE_WITH_KNOTS('',3,(#238901,#238902,#238903,#238904,#238905,
#238906,#238907,#238908,#238909,#238910,#238911,#238912,#238913,#238914,
#238915,#238916,#238917,#238918,#238919,#238920,#238921,#238922,#238923,
#238924,#238925,#238926,#238927,#238928,#238929,#238930,#238931,#238932,
#238933,#238934,#238935,#238936,#238937,#238938,#238939,#238940,#238941,
#238942,#238943,#238944,#238945,#238946,#238947,#238948,#238949,#238950,
#238951,#238952),.UNSPECIFIED.,.F.,.F.,(4,3,3,3,3,3,3,3,3,3,3,3,3,3,3,3,
3,4),(0.,2.58457451662736E-5,4.25394446196895E-5,6.46659869687634E-5,7.57292581433003E-5,
8.12608937305688E-5,8.26438026273859E-5,8.67925293178372E-5,0.000116015624426251,
0.000130188793976756,0.000151886926306215,0.000161963651211272,0.000162735992470945,
0.000173585058635674,0.000212487880462082,0.00025523817351434,0.000301397761152266,
0.000347170117271362),.UNSPECIFIED.);
#5177=B_SPLINE_CURVE_WITH_KNOTS('',3,(#238954,#238955,#238956,#238957,#238958,
#238959,#238960,#238961,#238962,#238963,#238964,#238965,#238966,#238967,
#238968,#238969,#238970,#238971,#238972,#238973,#238974,#238975,#238976,
#238977,#238978,#238979,#238980,#238981,#238982,#238983,#238984,#238985,
#238986,#238987,#238988,#238989,#238990,#238991,#238992,#238993,#238994,
#238995,#238996,#238997,#238998,#238999),.UNSPECIFIED.,.F.,.F.,(4,3,3,3,
3,3,3,3,3,3,3,3,3,3,3,4),(0.,2.57218162006404E-5,4.2156832256781E-5,6.45873314616977E-5,
7.58025810641561E-5,8.14102058653853E-5,8.28121120656925E-5,8.70178306666144E-5,
0.000116081955658562,0.000130526745999922,0.000162394111022053,0.000174035661333229,
0.000213138396956554,0.000256116935430458,0.000302406662851075,0.000348071322666458),
 .UNSPECIFIED.);
#5178=B_SPLINE_CURVE_WITH_KNOTS('',3,(#239000,#239001,#239002,#239003,#239004,
#239005,#239006,#239007,#239008,#239009,#239010,#239011,#239012,#239013,
#239014,#239015,#239016,#239017,#239018,#239019,#239020,#239021,#239022,
#239023,#239024,#239025,#239026,#239027,#239028,#239029,#239030,#239031,
#239032,#239033,#239034,#239035,#239036,#239037,#239038,#239039,#239040,
#239041,#239042,#239043,#239044,#239045,#239046,#239047,#239048,#239049,
#239050,#239051),.UNSPECIFIED.,.F.,.F.,(4,3,3,3,3,3,3,3,3,3,3,3,3,3,3,3,
3,4),(4.33680868994202E-19,4.29652152217032E-5,8.44519107624915E-5,0.000123669830876186,
0.000159788877370628,0.000170558847912619,0.000181218775907159,0.000181960046452394,
0.000214460062643333,0.000244755726197477,0.000255838271868938,0.000258503253867573,
0.00026108495517875,0.000289370476647778,0.000301101325502003,0.00032110951066363,
0.000331113603244443,0.000341117695825256),.UNSPECIFIED.);
#5179=B_SPLINE_CURVE_WITH_KNOTS('',3,(#239053,#239054,#239055,#239056,#239057,
#239058,#239059,#239060,#239061,#239062,#239063,#239064,#239065,#239066,
#239067,#239068,#239069,#239070,#239071,#239072,#239073,#239074,#239075,
#239076,#239077,#239078,#239079,#239080,#239081,#239082,#239083,#239084,
#239085,#239086,#239087,#239088,#239089,#239090,#239091,#239092,#239093,
#239094,#239095,#239096,#239097,#239098,#239099,#239100,#239101,#239102,
#239103,#239104),.UNSPECIFIED.,.F.,.F.,(4,3,3,3,3,3,3,3,3,3,3,3,3,3,3,3,
3,4),(1.73472347597681E-18,4.30706237865187E-5,8.47417087690789E-5,0.000124159989205212,
0.000160467076289721,0.000170998382116687,0.000182414994733761,0.000213747977645862,
0.000242415955903363,0.000256497573175038,0.000259169422895611,0.000261757777312417,
0.00028996513040298,0.000301877270772903,0.000321937017503145,0.000326951954185706,
0.000334474359209547,0.000341996764233388),.UNSPECIFIED.);
#5180=B_SPLINE_CURVE_WITH_KNOTS('',3,(#239105,#239106,#239107,#239108,#239109,
#239110,#239111,#239112,#239113,#239114,#239115,#239116,#239117,#239118,
#239119,#239120,#239121,#239122,#239123,#239124,#239125,#239126,#239127,
#239128,#239129,#239130,#239131,#239132,#239133,#239134,#239135,#239136,
#239137,#239138,#239139,#239140,#239141,#239142,#239143,#239144,#239145,
#239146,#239147,#239148,#239149,#239150,#239151,#239152,#239153,#239154,
#239155,#239156),.UNSPECIFIED.,.F.,.F.,(4,3,3,3,3,3,3,3,3,3,3,3,3,3,3,3,
3,4),(0.,2.5845745167758E-5,4.25394446195707E-5,6.46659869687025E-5,7.57292581432684E-5,
8.12608937305514E-5,8.26438026273721E-5,8.67925293178343E-5,0.000116015624427299,
0.000130188793976752,0.00015188692630621,0.000161963651211261,0.000162735992470939,
0.000173585058635669,0.000212487880461096,0.000255238173511359,0.000301397761144902,
0.000347170117271349),.UNSPECIFIED.);
#5181=B_SPLINE_CURVE_WITH_KNOTS('',3,(#239158,#239159,#239160,#239161,#239162,
#239163,#239164,#239165,#239166,#239167,#239168,#239169,#239170,#239171,
#239172,#239173,#239174,#239175,#239176,#239177,#239178,#239179,#239180,
#239181,#239182,#239183,#239184,#239185,#239186,#239187,#239188,#239189,
#239190,#239191,#239192,#239193,#239194,#239195,#239196,#239197,#239198,
#239199,#239200,#239201,#239202,#239203),.UNSPECIFIED.,.F.,.F.,(4,3,3,3,
3,3,3,3,3,3,3,3,3,3,3,4),(0.,2.57218162006442E-5,4.21568322567569E-5,6.45873314616859E-5,
7.58025810641504E-5,8.14102058653826E-5,8.28121120656907E-5,8.70178306666148E-5,
0.000116081955659045,0.000130526745999922,0.000162394111022048,0.00017403566133323,
0.000213138396959227,0.00025611693543571,0.000302406662858846,0.000348071322666472),
 .UNSPECIFIED.);
#5182=B_SPLINE_CURVE_WITH_KNOTS('',3,(#239204,#239205,#239206,#239207,#239208,
#239209,#239210,#239211,#239212,#239213,#239214,#239215,#239216,#239217,
#239218,#239219,#239220,#239221,#239222,#239223,#239224,#239225,#239226,
#239227,#239228,#239229,#239230,#239231,#239232,#239233,#239234,#239235,
#239236,#239237,#239238,#239239,#239240,#239241,#239242,#239243,#239244,
#239245,#239246,#239247,#239248,#239249,#239250,#239251,#239252,#239253,
#239254,#239255),.UNSPECIFIED.,.F.,.F.,(4,3,3,3,3,3,3,3,3,3,3,3,3,3,3,3,
3,4),(0.,4.29652152172934E-5,8.445191075492E-5,0.000123669830866065,0.000159788877357958,
0.000170558847912622,0.000181218775907161,0.000181960046452391,0.000214460062643236,
0.000244755726197423,0.000255838271868933,0.000258503253867568,0.000261084955178745,
0.000289370476648821,0.000301101325501995,0.00032110951066362,0.000331113603244432,
0.000341117695825244),.UNSPECIFIED.);
#5183=B_SPLINE_CURVE_WITH_KNOTS('',3,(#239257,#239258,#239259,#239260,#239261,
#239262,#239263,#239264,#239265,#239266,#239267,#239268,#239269,#239270,
#239271,#239272,#239273,#239274,#239275,#239276,#239277,#239278,#239279,
#239280,#239281,#239282,#239283,#239284,#239285,#239286,#239287,#239288,
#239289,#239290,#239291,#239292,#239293,#239294,#239295,#239296,#239297,
#239298,#239299,#239300,#239301,#239302,#239303,#239304,#239305,#239306,
#239307,#239308),.UNSPECIFIED.,.F.,.F.,(4,3,3,3,3,3,3,3,3,3,3,3,3,3,3,3,
3,4),(1.73472347597681E-18,4.30706237903578E-5,8.47417087758089E-5,0.000124159989214496,
0.000160467076301624,0.000170998382116703,0.000182414994733777,0.000213747977645874,
0.000242415955905344,0.000256497573175045,0.000259169422895618,0.000261757777312424,
0.000289965130400276,0.000301877270772905,0.000321937017503146,0.000326951954185706,
0.000334474359209547,0.000341996764233387),.UNSPECIFIED.);
#5184=B_SPLINE_CURVE_WITH_KNOTS('',3,(#239309,#239310,#239311,#239312,#239313,
#239314,#239315,#239316,#239317,#239318,#239319,#239320,#239321,#239322,
#239323,#239324,#239325,#239326,#239327,#239328,#239329,#239330,#239331,
#239332,#239333,#239334,#239335,#239336,#239337,#239338,#239339,#239340,
#239341,#239342,#239343,#239344,#239345,#239346,#239347,#239348,#239349,
#239350,#239351,#239352,#239353,#239354,#239355,#239356,#239357,#239358,
#239359,#239360),.UNSPECIFIED.,.F.,.F.,(4,3,3,3,3,3,3,3,3,3,3,3,3,3,3,3,
3,4),(0.,2.58457451683151E-5,4.25394446196292E-5,6.46659869687347E-5,7.57292581432875E-5,
8.12608937305638E-5,8.26438026273829E-5,8.67925293178402E-5,0.000116015624427729,
0.00013018879397676,0.00015188692630622,0.000161963651211276,0.00016273599247095,
0.00017358505863568,0.000212487880461049,0.000255238173512498,0.000301397761149868,
0.000347170117271345),.UNSPECIFIED.);
#5185=B_SPLINE_CURVE_WITH_KNOTS('',3,(#239362,#239363,#239364,#239365,#239366,
#239367,#239368,#239369,#239370,#239371,#239372,#239373,#239374,#239375,
#239376,#239377,#239378,#239379,#239380,#239381,#239382,#239383,#239384,
#239385,#239386,#239387,#239388,#239389,#239390,#239391,#239392,#239393,
#239394,#239395,#239396,#239397,#239398,#239399,#239400,#239401,#239402,
#239403,#239404,#239405,#239406,#239407),.UNSPECIFIED.,.F.,.F.,(4,3,3,3,
3,3,3,3,3,3,3,3,3,3,3,4),(0.,2.57218161996909E-5,4.21568322568114E-5,6.45873314617117E-5,
7.58025810641618E-5,8.14102058653869E-5,8.28121120656932E-5,8.7017830666612E-5,
0.000116081955658437,0.000130526745999918,0.000162394111022029,0.000174035661333224,
0.000213138396959559,0.000256116935436461,0.000302406662860391,0.000348071322666469),
 .UNSPECIFIED.);
#5186=B_SPLINE_CURVE_WITH_KNOTS('',3,(#239408,#239409,#239410,#239411,#239412,
#239413,#239414,#239415,#239416,#239417,#239418,#239419,#239420,#239421,
#239422,#239423,#239424,#239425,#239426,#239427,#239428,#239429,#239430,
#239431,#239432,#239433,#239434,#239435,#239436,#239437,#239438,#239439,
#239440,#239441,#239442,#239443,#239444,#239445,#239446,#239447,#239448,
#239449,#239450,#239451,#239452,#239453,#239454,#239455,#239456,#239457,
#239458,#239459),.UNSPECIFIED.,.F.,.F.,(4,3,3,3,3,3,3,3,3,3,3,3,3,3,3,3,
3,4),(0.,4.29652152190705E-5,8.44519107582359E-5,0.000123669830870871,0.000159788877364706,
0.000170558847912644,0.000181218775907184,0.000181960046452415,0.000214460062643127,
0.000244755726196831,0.000255838271868958,0.000258503253867592,0.00026108495517877,
0.000289370476648193,0.00030110132550202,0.000321109510663645,0.000331113603244458,
0.00034111769582527),.UNSPECIFIED.);
#5187=B_SPLINE_CURVE_WITH_KNOTS('',3,(#239461,#239462,#239463,#239464,#239465,
#239466,#239467,#239468,#239469,#239470,#239471,#239472,#239473,#239474,
#239475,#239476,#239477,#239478,#239479,#239480,#239481,#239482,#239483,
#239484,#239485,#239486,#239487,#239488,#239489,#239490,#239491,#239492,
#239493,#239494,#239495,#239496,#239497,#239498,#239499,#239500,#239501,
#239502,#239503,#239504,#239505,#239506,#239507,#239508,#239509,#239510,
#239511,#239512),.UNSPECIFIED.,.F.,.F.,(4,3,3,3,3,3,3,3,3,3,3,3,3,3,3,3,
3,4),(0.,4.30706237873028E-5,8.47417087702334E-5,0.00012415998920642,0.000160467076290766,
0.000170998382116705,0.000182414994733777,0.000213747977645876,0.000242415955903002,
0.000256497573175047,0.00025916942289562,0.000261757777312426,0.000289965130403416,
0.000301877270772908,0.000321937017503149,0.000326951954185709,0.000334474359209549,
0.00034199676423339),.UNSPECIFIED.);
#5188=B_SPLINE_CURVE_WITH_KNOTS('',3,(#239513,#239514,#239515,#239516,#239517,
#239518,#239519,#239520,#239521,#239522,#239523,#239524,#239525,#239526,
#239527,#239528,#239529,#239530,#239531,#239532,#239533,#239534,#239535,
#239536,#239537,#239538,#239539,#239540,#239541,#239542,#239543,#239544,
#239545,#239546,#239547,#239548,#239549,#239550,#239551,#239552,#239553,
#239554,#239555,#239556,#239557,#239558,#239559,#239560,#239561,#239562,
#239563,#239564),.UNSPECIFIED.,.F.,.F.,(4,3,3,3,3,3,3,3,3,3,3,3,3,3,3,3,
3,4),(0.,2.58457451661623E-5,4.25394446195541E-5,6.46659869686995E-5,7.57292581432722E-5,
8.12608937305585E-5,8.26438026273801E-5,8.67925293178448E-5,0.000116015624426535,
0.000130188793976767,0.000151886926306228,0.000161963651211281,0.000162735992470959,
0.00017358505863569,0.000212487880458905,0.000255238173506665,0.000301397761136841,
0.000347170117271379),.UNSPECIFIED.);
#5189=B_SPLINE_CURVE_WITH_KNOTS('',3,(#239566,#239567,#239568,#239569,#239570,
#239571,#239572,#239573,#239574,#239575,#239576,#239577,#239578,#239579,
#239580,#239581,#239582,#239583,#239584,#239585,#239586,#239587,#239588,
#239589,#239590,#239591,#239592,#239593,#239594,#239595,#239596,#239597,
#239598,#239599,#239600,#239601,#239602,#239603,#239604,#239605,#239606,
#239607,#239608,#239609,#239610,#239611),.UNSPECIFIED.,.F.,.F.,(4,3,3,3,
3,3,3,3,3,3,3,3,3,3,3,4),(0.,2.57218161991911E-5,4.21568322568509E-5,6.45873314617345E-5,
7.58025810641763E-5,8.14102058653972E-5,8.28121120657024E-5,8.70178306666181E-5,
0.000116081955657687,0.000130526745999927,0.000162394111022044,0.000174035661333236,
0.000213138396959808,0.000256116935436941,0.000302406662861117,0.000348071322666471),
 .UNSPECIFIED.);
#5190=B_SPLINE_CURVE_WITH_KNOTS('',3,(#239612,#239613,#239614,#239615,#239616,
#239617,#239618,#239619,#239620,#239621,#239622,#239623,#239624,#239625,
#239626,#239627,#239628,#239629,#239630,#239631,#239632,#239633,#239634,
#239635,#239636,#239637,#239638,#239639,#239640,#239641,#239642,#239643,
#239644,#239645,#239646,#239647,#239648,#239649,#239650,#239651,#239652,
#239653,#239654,#239655,#239656,#239657,#239658,#239659,#239660,#239661,
#239662,#239663),.UNSPECIFIED.,.F.,.F.,(4,3,3,3,3,3,3,3,3,3,3,3,3,3,3,3,
3,4),(4.33680868994202E-19,4.29652152163512E-5,8.44519107537964E-5,0.000123669830865421,
0.000159788877358528,0.000170558847912628,0.000181218775907168,0.000181960046452404,
0.000214460062643096,0.000244755726197257,0.000255838271868949,0.000258503253867584,
0.000261084955178762,0.000289370476649044,0.000301101325502016,0.000321109510663643,
0.000331113603244456,0.00034111769582527),.UNSPECIFIED.);
#5191=B_SPLINE_CURVE_WITH_KNOTS('',3,(#239665,#239666,#239667,#239668,#239669,
#239670,#239671,#239672,#239673,#239674,#239675,#239676,#239677,#239678,
#239679,#239680,#239681,#239682,#239683,#239684,#239685,#239686,#239687,
#239688,#239689,#239690,#239691,#239692,#239693,#239694,#239695,#239696,
#239697,#239698,#239699,#239700,#239701,#239702,#239703,#239704,#239705,
#239706,#239707,#239708,#239709,#239710,#239711,#239712,#239713,#239714,
#239715,#239716),.UNSPECIFIED.,.F.,.F.,(4,3,3,3,3,3,3,3,3,3,3,3,3,3,3,3,
3,4),(0.,4.30706237882266E-5,8.47417087718488E-5,0.000124159989208699,0.000160467076293763,
0.000170998382116694,0.00018241499473379,0.000213747977645869,0.000242415955902749,
0.000256497573175043,0.000259169422895617,0.000261757777312422,0.00028996513040296,
0.000301877270772907,0.00032193701750315,0.000326951954185711,0.000334474359209552,
0.000341996764233392),.UNSPECIFIED.);
#5192=B_SPLINE_CURVE_WITH_KNOTS('',3,(#239717,#239718,#239719,#239720,#239721,
#239722,#239723,#239724,#239725,#239726,#239727,#239728,#239729,#239730,
#239731,#239732,#239733,#239734,#239735,#239736,#239737,#239738,#239739,
#239740,#239741,#239742,#239743,#239744,#239745,#239746,#239747,#239748,
#239749,#239750,#239751,#239752,#239753,#239754,#239755,#239756,#239757,
#239758,#239759,#239760,#239761,#239762,#239763,#239764,#239765,#239766,
#239767,#239768),.UNSPECIFIED.,.F.,.F.,(4,3,3,3,3,3,3,3,3,3,3,3,3,3,3,3,
3,4),(0.,2.58457451676442E-5,4.25394446196521E-5,6.46659869687445E-5,7.57292581432907E-5,
8.12608937305638E-5,8.26438026273821E-5,8.67925293178369E-5,0.000116015624426859,
0.000130188793976755,0.000151886926306215,0.000161963651211276,0.000162735992470944,
0.000173585058635674,0.000212487880459347,0.000255238173508912,0.000301397761143805,
0.000347170117271363),.UNSPECIFIED.);
#5193=B_SPLINE_CURVE_WITH_KNOTS('',3,(#239770,#239771,#239772,#239773,#239774,
#239775,#239776,#239777,#239778,#239779,#239780,#239781,#239782,#239783,
#239784,#239785,#239786,#239787,#239788,#239789,#239790,#239791,#239792,
#239793,#239794,#239795,#239796,#239797,#239798,#239799,#239800,#239801,
#239802,#239803,#239804,#239805,#239806,#239807,#239808,#239809,#239810,
#239811,#239812,#239813,#239814,#239815),.UNSPECIFIED.,.F.,.F.,(4,3,3,3,
3,3,3,3,3,3,3,3,3,3,3,4),(6.95243322195995E-18,2.57218161995218E-5,4.21568322569579E-5,
6.45873314617886E-5,7.58025810642039E-5,8.14102058654115E-5,8.28121120657135E-5,
8.70178306666192E-5,0.000116081955659034,0.000130526745999925,0.000162394111022051,
0.000174035661333231,0.000213138396961045,0.000256116935439446,0.00030240666286506,
0.000348071322666456),.UNSPECIFIED.);
#5194=B_SPLINE_CURVE_WITH_KNOTS('',3,(#239816,#239817,#239818,#239819,#239820,
#239821,#239822,#239823,#239824,#239825,#239826,#239827,#239828,#239829,
#239830,#239831,#239832,#239833,#239834,#239835,#239836,#239837,#239838,
#239839,#239840,#239841,#239842,#239843,#239844,#239845,#239846,#239847,
#239848,#239849,#239850,#239851,#239852,#239853,#239854,#239855,#239856,
#239857,#239858,#239859,#239860,#239861,#239862,#239863,#239864,#239865,
#239866,#239867),.UNSPECIFIED.,.F.,.F.,(4,3,3,3,3,3,3,3,3,3,3,3,3,3,3,3,
3,4),(0.,4.29652152161983E-5,8.44519107532164E-5,0.00012366983086397,0.000159788877355752,
0.000170558847912625,0.000181218775907166,0.000181960046452406,0.000214460062642528,
0.000244755726195342,0.000255838271868948,0.000258503253867583,0.000261084955178761,
0.000289370476648543,0.000301101325502016,0.000321109510663643,0.000331113603244457,
0.000341117695825271),.UNSPECIFIED.);
#5195=B_SPLINE_CURVE_WITH_KNOTS('',3,(#239869,#239870,#239871,#239872,#239873,
#239874,#239875,#239876,#239877,#239878,#239879,#239880,#239881,#239882,
#239883,#239884,#239885,#239886,#239887,#239888,#239889,#239890,#239891,
#239892,#239893,#239894,#239895,#239896,#239897,#239898,#239899,#239900,
#239901,#239902,#239903,#239904,#239905,#239906,#239907,#239908,#239909,
#239910,#239911,#239912,#239913,#239914,#239915,#239916,#239917,#239918,
#239919,#239920),.UNSPECIFIED.,.F.,.F.,(4,3,3,3,3,3,3,3,3,3,3,3,3,3,3,3,
3,4),(0.,4.30706237856902E-5,8.47417087673733E-5,0.00012415998920248,0.000160467076285652,
0.000170998382116697,0.000182414994733777,0.000213747977645874,0.000242415955903854,
0.00025649757317505,0.000259169422895623,0.000261757777312429,0.000289965130402078,
0.000301877270772916,0.000321937017503159,0.00032695195418572,0.000334474359209561,
0.000341996764233403),.UNSPECIFIED.);
#5196=B_SPLINE_CURVE_WITH_KNOTS('',3,(#239921,#239922,#239923,#239924,#239925,
#239926,#239927,#239928,#239929,#239930,#239931,#239932,#239933,#239934,
#239935,#239936,#239937,#239938,#239939,#239940,#239941,#239942,#239943,
#239944,#239945,#239946,#239947,#239948,#239949,#239950,#239951,#239952,
#239953,#239954,#239955,#239956,#239957,#239958,#239959,#239960,#239961,
#239962,#239963,#239964,#239965,#239966,#239967,#239968,#239969,#239970,
#239971,#239972),.UNSPECIFIED.,.F.,.F.,(4,3,3,3,3,3,3,3,3,3,3,3,3,3,3,3,
3,4),(3.46944695195361E-18,2.58457451684559E-5,4.25394446196587E-5,6.46659869687525E-5,
7.57292581432994E-5,8.12608937305728E-5,8.26438026273912E-5,8.67925293178463E-5,
0.000116015624427615,0.000130188793976768,0.000151886926306228,0.000161963651211276,
0.000162735992470959,0.000173585058635689,0.000212487880459735,0.000255238173508576,
0.000301397761140788,0.000347170117271376),.UNSPECIFIED.);
#5197=B_SPLINE_CURVE_WITH_KNOTS('',3,(#239974,#239975,#239976,#239977,#239978,
#239979,#239980,#239981,#239982,#239983,#239984,#239985,#239986,#239987,
#239988,#239989,#239990,#239991,#239992,#239993,#239994,#239995,#239996,
#239997,#239998,#239999,#240000,#240001,#240002,#240003,#240004,#240005,
#240006,#240007,#240008,#240009,#240010,#240011,#240012,#240013,#240014,
#240015,#240016,#240017,#240018,#240019),.UNSPECIFIED.,.F.,.F.,(4,3,3,3,
3,3,3,3,3,3,3,3,3,3,3,4),(0.,2.5721816198903E-5,4.21568322569722E-5,6.45873314617926E-5,
7.58025810642029E-5,8.1410205865408E-5,8.28121120657092E-5,8.70178306666131E-5,
0.000116081955658234,0.00013052674599992,0.000162394111022023,0.000174035661333226,
0.000213138396959779,0.000256116935436934,0.000302406662861205,0.000348071322666452),
 .UNSPECIFIED.);
#5198=B_SPLINE_CURVE_WITH_KNOTS('',3,(#240020,#240021,#240022,#240023,#240024,
#240025,#240026,#240027,#240028,#240029,#240030,#240031,#240032,#240033,
#240034,#240035,#240036,#240037,#240038,#240039,#240040,#240041,#240042,
#240043,#240044,#240045,#240046,#240047,#240048,#240049,#240050,#240051,
#240052,#240053,#240054,#240055,#240056,#240057,#240058,#240059,#240060,
#240061,#240062,#240063,#240064,#240065,#240066,#240067,#240068,#240069,
#240070,#240071),.UNSPECIFIED.,.F.,.F.,(4,3,3,3,3,3,3,3,3,3,3,3,3,3,3,3,
3,4),(4.33680868994202E-19,4.29652152147306E-5,8.4451910751015E-5,0.000123669830861697,
0.00015978887735388,0.000170558847912629,0.000181218775907168,0.000181960046452407,
0.000214460062643719,0.000244755726198878,0.000255838271868943,0.000258503253867578,
0.000261084955178756,0.000289370476647109,0.000301101325502007,0.000321109510663632,
0.000331113603244445,0.000341117695825258),.UNSPECIFIED.);
#5199=B_SPLINE_CURVE_WITH_KNOTS('',3,(#240073,#240074,#240075,#240076,#240077,
#240078,#240079,#240080,#240081,#240082,#240083,#240084,#240085,#240086,
#240087,#240088,#240089,#240090,#240091,#240092,#240093,#240094,#240095,
#240096,#240097,#240098,#240099,#240100,#240101,#240102,#240103,#240104,
#240105,#240106,#240107,#240108,#240109,#240110,#240111,#240112,#240113,
#240114,#240115,#240116,#240117,#240118,#240119,#240120,#240121,#240122,
#240123,#240124),.UNSPECIFIED.,.F.,.F.,(4,3,3,3,3,3,3,3,3,3,3,3,3,3,3,3,
3,4),(0.,4.30706237868881E-5,8.4741708769574E-5,0.000124159989205557,0.000160467076289722,
0.000170998382116688,0.000182414994733766,0.000213747977645864,0.000242415955901617,
0.000256497573175039,0.000259169422895613,0.000261757777312418,0.000289965130404738,
0.000301877270772905,0.000321937017503148,0.000326951954185709,0.00033447435920955,
0.000341996764233391),.UNSPECIFIED.);
#5200=B_SPLINE_CURVE_WITH_KNOTS('',3,(#240125,#240126,#240127,#240128,#240129,
#240130,#240131,#240132,#240133,#240134,#240135,#240136,#240137,#240138,
#240139,#240140,#240141,#240142,#240143,#240144,#240145,#240146,#240147,
#240148,#240149,#240150,#240151,#240152,#240153,#240154,#240155,#240156,
#240157,#240158,#240159,#240160,#240161,#240162,#240163,#240164,#240165,
#240166,#240167,#240168,#240169,#240170,#240171,#240172,#240173,#240174,
#240175,#240176),.UNSPECIFIED.,.F.,.F.,(4,3,3,3,3,3,3,3,3,3,3,3,3,3,3,3,
3,4),(3.46944695195361E-18,2.58457451686505E-5,4.25394446196537E-5,6.46659869687495E-5,
7.57292581432974E-5,8.12608937305713E-5,8.26438026273898E-5,8.67925293178453E-5,
0.000116015624427858,0.000130188793976766,0.000151886926306227,0.000161963651211277,
0.000162735992470957,0.000173585058635687,0.000212487880459702,0.000255238173508743,
0.000301397761141439,0.000347170117271355),.UNSPECIFIED.);
#5201=B_SPLINE_CURVE_WITH_KNOTS('',3,(#240178,#240179,#240180,#240181,#240182,
#240183,#240184,#240185,#240186,#240187,#240188,#240189,#240190,#240191,
#240192,#240193,#240194,#240195,#240196,#240197,#240198,#240199,#240200,
#240201,#240202,#240203,#240204,#240205,#240206,#240207,#240208,#240209,
#240210,#240211,#240212,#240213,#240214,#240215,#240216,#240217,#240218,
#240219,#240220,#240221,#240222,#240223),.UNSPECIFIED.,.F.,.F.,(4,3,3,3,
3,3,3,3,3,3,3,3,3,3,3,4),(0.,2.57218162003092E-5,4.21568322568195E-5,6.45873314617163E-5,
7.58025810641646E-5,8.14102058653888E-5,8.28121120656949E-5,8.7017830666613E-5,
0.000116081955658734,0.00013052674599992,0.000162394111022031,0.000174035661333226,
0.000213138396957737,0.000256116935432863,0.000302406662854935,0.000348071322666467),
 .UNSPECIFIED.);
#5202=B_SPLINE_CURVE_WITH_KNOTS('',3,(#240224,#240225,#240226,#240227,#240228,
#240229,#240230,#240231,#240232,#240233,#240234,#240235,#240236,#240237,
#240238,#240239,#240240,#240241,#240242,#240243,#240244,#240245,#240246,
#240247,#240248,#240249,#240250,#240251,#240252,#240253,#240254,#240255,
#240256,#240257,#240258,#240259,#240260,#240261,#240262,#240263,#240264,
#240265,#240266,#240267,#240268,#240269,#240270,#240271,#240272,#240273,
#240274,#240275),.UNSPECIFIED.,.F.,.F.,(4,3,3,3,3,3,3,3,3,3,3,3,3,3,3,3,
3,4),(0.,4.29652152126629E-5,8.44519107479425E-5,0.000123669830858356,0.000159788877350821,
0.000170558847912639,0.000181218775907178,0.000181960046452419,0.000214460062643348,
0.000244755726197514,0.000255838271868955,0.00025850325386759,0.000261084955178767,
0.000289370476647847,0.000301101325502019,0.000321109510663645,0.000331113603244458,
0.000341117695825271),.UNSPECIFIED.);
#5203=B_SPLINE_CURVE_WITH_KNOTS('',3,(#240277,#240278,#240279,#240280,#240281,
#240282,#240283,#240284,#240285,#240286,#240287,#240288,#240289,#240290,
#240291,#240292,#240293,#240294,#240295,#240296,#240297,#240298,#240299,
#240300,#240301,#240302,#240303,#240304,#240305,#240306,#240307,#240308,
#240309,#240310,#240311,#240312,#240313,#240314,#240315,#240316,#240317,
#240318,#240319,#240320,#240321,#240322,#240323,#240324,#240325,#240326,
#240327,#240328),.UNSPECIFIED.,.F.,.F.,(4,3,3,3,3,3,3,3,3,3,3,3,3,3,3,3,
3,4),(8.67361737988403E-19,4.30706237870993E-5,8.47417087698459E-5,0.000124159989205834,
0.000160467076289949,0.000170998382116697,0.000182414994733785,0.000213747977645869,
0.0002424159559032,0.00025649757317504,0.000259169422895614,0.000261757777312419,
0.000289965130403263,0.000301877270772901,0.000321937017503143,0.000326951954185703,
0.000334474359209543,0.000341996764233384),.UNSPECIFIED.);
#5204=B_SPLINE_CURVE_WITH_KNOTS('',3,(#240329,#240330,#240331,#240332,#240333,
#240334,#240335,#240336,#240337,#240338,#240339,#240340,#240341,#240342,
#240343,#240344,#240345,#240346,#240347,#240348,#240349,#240350,#240351,
#240352,#240353,#240354,#240355,#240356,#240357,#240358,#240359,#240360,
#240361,#240362,#240363,#240364,#240365,#240366,#240367,#240368,#240369,
#240370,#240371,#240372,#240373,#240374,#240375,#240376,#240377,#240378,
#240379,#240380),.UNSPECIFIED.,.F.,.F.,(4,3,3,3,3,3,3,3,3,3,3,3,3,3,3,3,
3,4),(0.,2.58457451673367E-5,4.25394446196646E-5,6.46659869687537E-5,7.57292581432982E-5,
8.12608937305705E-5,8.26438026273886E-5,8.67925293178428E-5,0.000116015624426733,
0.000130188793976764,0.000151886926306225,0.000161963651211275,0.000162735992470955,
0.000173585058635686,0.000212487880457774,0.000255238173504083,0.0003013977611323,
0.00034717011727137),.UNSPECIFIED.);
#5205=B_SPLINE_CURVE_WITH_KNOTS('',3,(#240382,#240383,#240384,#240385,#240386,
#240387,#240388,#240389,#240390,#240391,#240392,#240393,#240394,#240395,
#240396,#240397,#240398,#240399,#240400,#240401,#240402,#240403,#240404,
#240405,#240406,#240407,#240408,#240409,#240410,#240411,#240412,#240413,
#240414,#240415,#240416,#240417,#240418,#240419,#240420,#240421,#240422,
#240423,#240424,#240425,#240426,#240427),.UNSPECIFIED.,.F.,.F.,(4,3,3,3,
3,3,3,3,3,3,3,3,3,3,3,4),(0.,2.57218162008265E-5,4.21568322568929E-5,6.45873314617525E-5,
7.58025810641823E-5,8.14102058653972E-5,8.28121120657009E-5,8.70178306666121E-5,
0.000116081955659349,0.000130526745999918,0.000162394111022029,0.000174035661333224,
0.000213138396959796,0.00025611693543712,0.000302406662862035,0.000348071322666464),
 .UNSPECIFIED.);
#5206=B_SPLINE_CURVE_WITH_KNOTS('',3,(#240428,#240429,#240430,#240431,#240432,
#240433,#240434,#240435,#240436,#240437,#240438,#240439,#240440,#240441,
#240442,#240443,#240444,#240445,#240446,#240447,#240448,#240449,#240450,
#240451,#240452,#240453,#240454,#240455,#240456,#240457,#240458,#240459,
#240460,#240461,#240462,#240463,#240464,#240465,#240466,#240467,#240468,
#240469,#240470,#240471,#240472,#240473,#240474,#240475,#240476,#240477,
#240478,#240479),.UNSPECIFIED.,.F.,.F.,(4,3,3,3,3,3,3,3,3,3,3,3,3,3,3,3,
3,4),(0.,4.29652152136727E-5,8.44519107495488E-5,0.000123669830860388,0.000159788877352989,
0.000170558847912636,0.000181218775907175,0.000181960046452406,0.000214460062643941,
0.000244755726199492,0.000255838271868946,0.00025850325386758,0.000261084955178758,
0.000289370476647275,0.000301101325502007,0.000321109510663631,0.000331113603244443,
0.000341117695825255),.UNSPECIFIED.);
#5207=B_SPLINE_CURVE_WITH_KNOTS('',3,(#240481,#240482,#240483,#240484,#240485,
#240486,#240487,#240488,#240489,#240490,#240491,#240492,#240493,#240494,
#240495,#240496,#240497,#240498,#240499,#240500,#240501,#240502,#240503,
#240504,#240505,#240506,#240507,#240508,#240509,#240510,#240511,#240512,
#240513,#240514,#240515,#240516,#240517,#240518,#240519,#240520,#240521,
#240522,#240523,#240524,#240525,#240526,#240527,#240528,#240529,#240530,
#240531,#240532),.UNSPECIFIED.,.F.,.F.,(4,3,3,3,3,3,3,3,3,3,3,3,3,3,3,3,
3,4),(1.22969749649977E-17,4.30706237866378E-5,8.47417087689707E-5,0.000124159989204571,
0.000160467076288245,0.000170998382116699,0.000182414994733777,0.000213747977645869,
0.000242415955902751,0.000256497573175039,0.000259169422895612,0.000261757777312417,
0.000289965130403974,0.000301877270772898,0.000321937017503138,0.000326951954185699,
0.000334474359209539,0.000341996764233379),.UNSPECIFIED.);
#5208=B_SPLINE_CURVE_WITH_KNOTS('',3,(#240533,#240534,#240535,#240536,#240537,
#240538,#240539,#240540,#240541,#240542,#240543,#240544,#240545,#240546,
#240547,#240548,#240549,#240550,#240551,#240552,#240553,#240554,#240555,
#240556,#240557,#240558,#240559,#240560,#240561,#240562,#240563,#240564,
#240565,#240566,#240567,#240568,#240569,#240570,#240571,#240572,#240573,
#240574,#240575,#240576,#240577,#240578,#240579,#240580,#240581,#240582,
#240583,#240584),.UNSPECIFIED.,.F.,.F.,(4,3,3,3,3,3,3,3,3,3,3,3,3,3,3,3,
3,4),(0.,2.58457451669027E-5,4.25394446195448E-5,6.46659869686927E-5,7.57292581432667E-5,
8.12608937305537E-5,8.26438026273754E-5,8.67925293178407E-5,0.000116015624426837,
0.000130188793976761,0.000151886926306221,0.000161963651211277,0.000162735992470951,
0.000173585058635681,0.000212487880459692,0.0002552381735098,0.000301397761145626,
0.000347170117271346),.UNSPECIFIED.);
#5209=B_SPLINE_CURVE_WITH_KNOTS('',3,(#240586,#240587,#240588,#240589,#240590,
#240591,#240592,#240593,#240594,#240595,#240596,#240597,#240598,#240599,
#240600,#240601,#240602,#240603,#240604,#240605,#240606,#240607,#240608,
#240609,#240610,#240611,#240612,#240613,#240614,#240615,#240616,#240617,
#240618,#240619,#240620,#240621,#240622,#240623,#240624,#240625,#240626,
#240627,#240628,#240629,#240630,#240631),.UNSPECIFIED.,.F.,.F.,(4,3,3,3,
3,3,3,3,3,3,3,3,3,3,3,4),(0.,2.5721816200257E-5,4.21568322568039E-5,6.45873314617086E-5,
7.5802581064161E-5,8.14102058653872E-5,8.28121120656937E-5,8.70178306666133E-5,
0.000116081955658472,0.00013052674599992,0.000162394111022039,0.000174035661333227,
0.000213138396957767,0.000256116935432745,0.000302406662854146,0.00034807132266647),
 .UNSPECIFIED.);
#5210=B_SPLINE_CURVE_WITH_KNOTS('',3,(#240632,#240633,#240634,#240635,#240636,
#240637,#240638,#240639,#240640,#240641,#240642,#240643,#240644,#240645,
#240646,#240647,#240648,#240649,#240650,#240651,#240652,#240653,#240654,
#240655,#240656,#240657,#240658,#240659,#240660,#240661,#240662,#240663,
#240664,#240665,#240666,#240667,#240668,#240669,#240670,#240671,#240672,
#240673,#240674,#240675,#240676,#240677,#240678,#240679,#240680,#240681,
#240682,#240683),.UNSPECIFIED.,.F.,.F.,(4,3,3,3,3,3,3,3,3,3,3,3,3,3,3,3,
3,4),(4.33680868994202E-19,4.2965215214098E-5,8.44519107505796E-5,0.000123669830862313,
0.000159788877356241,0.000170558847912639,0.000181218775907178,0.000181960046452412,
0.000214460062644004,0.000244755726199407,0.000255838271868955,0.000258503253867589,
0.000261084955178767,0.000289370476646998,0.000301101325502019,0.000321109510663644,
0.000331113603244457,0.00034111769582527),.UNSPECIFIED.);
#5211=B_SPLINE_CURVE_WITH_KNOTS('',3,(#240685,#240686,#240687,#240688,#240689,
#240690,#240691,#240692,#240693,#240694,#240695,#240696,#240697,#240698,
#240699,#240700,#240701,#240702,#240703,#240704,#240705,#240706,#240707,
#240708,#240709,#240710,#240711,#240712,#240713,#240714,#240715,#240716,
#240717,#240718,#240719,#240720,#240721,#240722,#240723,#240724,#240725,
#240726,#240727,#240728,#240729,#240730,#240731,#240732,#240733,#240734,
#240735,#240736),.UNSPECIFIED.,.F.,.F.,(4,3,3,3,3,3,3,3,3,3,3,3,3,3,3,3,
3,4),(0.,4.30706237867457E-5,8.47417087691177E-5,0.00012415998920471,0.000160467076288282,
0.000170998382116703,0.000182414994733785,0.000213747977645875,0.00024241595590493,
0.000256497573175048,0.000259169422895621,0.000261757777312427,0.000289965130402185,
0.000301877270772907,0.000321937017503147,0.000326951954185707,0.000334474359209547,
0.000341996764233387),.UNSPECIFIED.);
#5212=B_SPLINE_CURVE_WITH_KNOTS('',3,(#240737,#240738,#240739,#240740,#240741,
#240742,#240743,#240744,#240745,#240746,#240747,#240748,#240749,#240750,
#240751,#240752,#240753,#240754,#240755,#240756,#240757,#240758,#240759,
#240760,#240761,#240762,#240763,#240764,#240765,#240766,#240767,#240768,
#240769,#240770,#240771,#240772,#240773,#240774,#240775,#240776,#240777,
#240778,#240779,#240780,#240781,#240782,#240783,#240784,#240785,#240786,
#240787,#240788),.UNSPECIFIED.,.F.,.F.,(4,3,3,3,3,3,3,3,3,3,3,3,3,3,3,3,
3,4),(0.,2.58457451683501E-5,4.25394446195563E-5,6.46659869686992E-5,7.57292581432707E-5,
8.12608937305565E-5,8.26438026273779E-5,8.67925293178422E-5,0.000116015624427275,
0.000130188793976763,0.000151886926306224,0.000161963651211262,0.000162735992470954,
0.000173585058635684,0.000212487880461338,0.000255238173512569,0.000301397761148645,
0.000347170117271369),.UNSPECIFIED.);
#5213=B_SPLINE_CURVE_WITH_KNOTS('',3,(#240790,#240791,#240792,#240793,#240794,
#240795,#240796,#240797,#240798,#240799,#240800,#240801,#240802,#240803,
#240804,#240805,#240806,#240807,#240808,#240809,#240810,#240811,#240812,
#240813,#240814,#240815,#240816,#240817,#240818,#240819,#240820,#240821,
#240822,#240823,#240824,#240825,#240826,#240827,#240828,#240829,#240830,
#240831,#240832,#240833,#240834,#240835),.UNSPECIFIED.,.F.,.F.,(4,3,3,3,
3,3,3,3,3,3,3,3,3,3,3,4),(0.,2.57218161991932E-5,4.21568322567385E-5,6.45873314616776E-5,
7.58025810641472E-5,8.1410205865382E-5,8.28121120656907E-5,8.70178306666167E-5,
0.00011608195565819,0.000130526745999925,0.00016239411102205,0.000174035661333233,
0.000213138396959465,0.00025611693543621,0.00030240666285981,0.000348071322666468),
 .UNSPECIFIED.);
#5214=B_SPLINE_CURVE_WITH_KNOTS('',3,(#240836,#240837,#240838,#240839,#240840,
#240841,#240842,#240843,#240844,#240845,#240846,#240847,#240848,#240849,
#240850,#240851,#240852,#240853,#240854,#240855,#240856,#240857,#240858,
#240859,#240860,#240861,#240862,#240863,#240864,#240865,#240866,#240867,
#240868,#240869,#240870,#240871,#240872,#240873,#240874,#240875,#240876,
#240877,#240878,#240879,#240880,#240881,#240882,#240883,#240884,#240885,
#240886,#240887),.UNSPECIFIED.,.F.,.F.,(4,3,3,3,3,3,3,3,3,3,3,3,3,3,3,3,
3,4),(0.,4.29652152176409E-5,8.44519107557594E-5,0.000123669830867554,0.000159788877360428,
0.000170558847912633,0.000181218775907172,0.000181960046452405,0.000214460062643479,
0.000244755726198168,0.000255838271868949,0.000258503253867584,0.000261084955178762,
0.000289370476647912,0.000301101325502014,0.00032110951066364,0.000331113603244453,
0.000341117695825266),.UNSPECIFIED.);
#5215=B_SPLINE_CURVE_WITH_KNOTS('',3,(#253551,#253552,#253553,#253554),
 .UNSPECIFIED.,.F.,.F.,(4,4),(1.73472347597681E-17,0.000497709506657957),
 .UNSPECIFIED.);
#5216=B_SPLINE_CURVE_WITH_KNOTS('',3,(#253556,#253557,#253558,#253559,#253560,
#253561,#253562,#253563,#253564,#253565,#253566,#253567,#253568,#253569,
#253570,#253571,#253572,#253573,#253574,#253575,#253576,#253577),
 .UNSPECIFIED.,.F.,.F.,(4,2,2,2,2,2,2,2,2,2,4),(0.000497709506657957,0.000958469059060371,
0.00141922861146278,0.0018799881638652,0.0021103679400664,0.0021679628841167,
0.00219676035614186,0.00222555782816702,0.00225435530019218,0.00228315277221733,
0.00234074771626765),.UNSPECIFIED.);
#5217=B_SPLINE_CURVE_WITH_KNOTS('',3,(#253583,#253584,#253585,#253586,#253587,
#253588,#253589,#253590,#253591,#253592,#253593,#253594,#253595,#253596,
#253597,#253598,#253599,#253600,#253601,#253602,#253603,#253604),
 .UNSPECIFIED.,.F.,.F.,(4,2,2,2,2,2,2,2,2,2,4),(1.9871740492849E-9,5.85234868205088E-5,
8.77842366437273E-5,0.000117044986466946,0.000146305736290164,0.000175566486113383,
0.000234087985759818,0.000468173984345514,0.000936345981516908,0.0014045179786883,
0.00187268997585969),.UNSPECIFIED.);
#5218=B_SPLINE_CURVE_WITH_KNOTS('',3,(#253606,#253607,#253608,#253609,#253610,
#253611,#253612,#253613,#253614,#253615,#253616,#253617,#253618,#253619,
#253620,#253621,#253622,#253623,#253624,#253625,#253626,#253627),
 .UNSPECIFIED.,.F.,.F.,(4,3,3,3,3,3,3,4),(0.00187268997585969,0.00199834274779399,
0.00204546253726935,0.00208669235306029,0.00220550294837832,0.00223099670832857,
0.00230314888596272,0.00237530106359686),.UNSPECIFIED.);
#5219=B_SPLINE_CURVE_WITH_KNOTS('',3,(#253635,#253636,#253637,#253638),
 .UNSPECIFIED.,.F.,.F.,(4,4),(3.46944695195361E-18,0.000776824705292371),
 .UNSPECIFIED.);
#5220=B_SPLINE_CURVE_WITH_KNOTS('',3,(#253640,#253641,#253642,#253643),
 .UNSPECIFIED.,.F.,.F.,(4,4),(0.,0.000776824705292379),.UNSPECIFIED.);
#5221=B_SPLINE_CURVE_WITH_KNOTS('',3,(#253682,#253683,#253684,#253685,#253686,
#253687,#253688,#253689,#253690,#253691),.UNSPECIFIED.,.F.,.F.,(4,3,3,4),
(0.00224752972328446,0.00254000000002921,0.0127000000034794,0.0252059134417286),
 .UNSPECIFIED.);
#5222=B_SPLINE_CURVE_WITH_KNOTS('',3,(#253695,#253696,#253697,#253698),
 .UNSPECIFIED.,.F.,.F.,(4,4),(-1.43540833573195E-5,0.000600070195786084),
 .UNSPECIFIED.);
#5223=B_SPLINE_CURVE_WITH_KNOTS('',3,(#253700,#253701,#253702,#253703,#253704,
#253705,#253706,#253707,#253708,#253709,#253710,#253711,#253712,#253713,
#253714,#253715,#253716,#253717,#253718,#253719,#253720,#253721,#253722,
#253723,#253724,#253725,#253726,#253727,#253728,#253729,#253730,#253731,
#253732,#253733,#253734,#253735,#253736,#253737,#253738,#253739,#253740,
#253741,#253742,#253743,#253744,#253745,#253746,#253747,#253748,#253749,
#253750,#253751,#253752,#253753,#253754),.UNSPECIFIED.,.F.,.F.,(4,3,3,3,
3,3,3,3,3,3,3,3,3,3,3,3,3,3,4),(0.000110053346854241,0.000527311723102858,
0.000718200211016914,0.000854122275949536,0.00126501374481543,0.00132634707517959,
0.00168651061235045,0.00193449393934226,0.00222985612775647,0.00251426340799128,
0.00254264080350493,0.00300412786917268,0.00333765384253305,0.00375893453183028,
0.00409210357716868,0.00415888746486257,0.00449321052526377,0.00480933253535804,
0.00497522826015563),.UNSPECIFIED.);
#5224=B_SPLINE_CURVE_WITH_KNOTS('',3,(#253758,#253759,#253760,#253761,#253762,
#253763,#253764,#253765,#253766,#253767,#253768,#253769,#253770,#253771,
#253772,#253773,#253774,#253775,#253776,#253777,#253778,#253779,#253780,
#253781,#253782,#253783,#253784,#253785,#253786,#253787,#253788,#253789,
#253790,#253791,#253792,#253793,#253794,#253795,#253796,#253797,#253798,
#253799,#253800,#253801,#253802,#253803,#253804,#253805,#253806),
 .UNSPECIFIED.,.F.,.F.,(4,3,3,3,3,3,3,3,3,3,3,3,3,3,3,3,4),(0.,0.000552804620400313,
0.000807500349755513,0.0012059666217394,0.00162007673419067,0.0021864702767717,
0.00241193324347881,0.00243219312565017,0.00283904062399015,0.00315006133501463,
0.0032484770180594,0.00361789986521821,0.00391885772791828,0.00407541417390928,
0.00422088317608792,0.00461166893086815,0.00482386648695763),
 .UNSPECIFIED.);
#5225=B_SPLINE_CURVE_WITH_KNOTS('',3,(#253807,#253808,#253809,#253810),
 .UNSPECIFIED.,.F.,.F.,(4,4),(6.04918746141641E-17,0.000614424279130608),
 .UNSPECIFIED.);
#5226=B_SPLINE_CURVE_WITH_KNOTS('',3,(#253812,#253813,#253814,#253815),
 .UNSPECIFIED.,.F.,.F.,(4,4),(-1.43540833568566E-5,0.000600070195786399),
 .UNSPECIFIED.);
#5227=B_SPLINE_CURVE_WITH_KNOTS('',3,(#253817,#253818,#253819,#253820,#253821,
#253822,#253823,#253824,#253825,#253826,#253827,#253828,#253829,#253830,
#253831,#253832,#253833,#253834,#253835,#253836,#253837,#253838,#253839,
#253840,#253841,#253842,#253843,#253844,#253845,#253846,#253847,#253848,
#253849,#253850,#253851,#253852,#253853,#253854,#253855,#253856,#253857,
#253858,#253859,#253860,#253861,#253862,#253863,#253864,#253865,#253866,
#253867,#253868,#253869,#253870,#253871),.UNSPECIFIED.,.F.,.F.,(4,3,3,3,
3,3,3,3,3,3,3,3,3,3,3,3,3,3,4),(0.000110053346854265,0.000527311723250969,
0.000718200211016931,0.000854122275951405,0.00126501374442658,0.0013263470751796,
0.00168651061235195,0.00193449393934226,0.00222985612779087,0.0025142634079924,
0.00254264080350493,0.00300412786893507,0.00333765384253336,0.00375893453183026,
0.00409210357719457,0.00415888746486208,0.00449321052529187,0.0048093325354323,
0.00497522826015559),.UNSPECIFIED.);
#5228=B_SPLINE_CURVE_WITH_KNOTS('',3,(#253875,#253876,#253877,#253878,#253879,
#253880,#253881,#253882,#253883,#253884,#253885,#253886,#253887,#253888,
#253889,#253890,#253891,#253892,#253893,#253894,#253895,#253896,#253897,
#253898,#253899,#253900,#253901,#253902,#253903,#253904,#253905,#253906,
#253907,#253908,#253909,#253910,#253911,#253912,#253913,#253914,#253915,
#253916,#253917,#253918,#253919,#253920,#253921,#253922,#253923),
 .UNSPECIFIED.,.F.,.F.,(4,3,3,3,3,3,3,3,3,3,3,3,3,3,3,3,4),(0.,0.000552804620158884,
0.000807500349754644,0.00120596662173943,0.00162007673419057,0.00218647027534087,
0.00241193324347885,0.00243219312565013,0.00283904062398887,0.00315006133493916,
0.00324847701805844,0.00361789986521828,0.00391885772791061,0.00407541417390921,
0.00422088317608798,0.00461166893084222,0.00482386648695769),
 .UNSPECIFIED.);
#5229=B_SPLINE_CURVE_WITH_KNOTS('',3,(#253925,#253926,#253927,#253928),
 .UNSPECIFIED.,.F.,.F.,(4,4),(1.47196168001604E-17,0.000614424279130721),
 .UNSPECIFIED.);
#5230=B_SPLINE_CURVE_WITH_KNOTS('',3,(#253932,#253933,#253934,#253935),
 .UNSPECIFIED.,.F.,.F.,(4,4),(-1.43540833566919E-5,0.000600070195786593),
 .UNSPECIFIED.);
#5231=B_SPLINE_CURVE_WITH_KNOTS('',3,(#253937,#253938,#253939,#253940,#253941,
#253942,#253943,#253944,#253945,#253946,#253947,#253948,#253949,#253950,
#253951,#253952,#253953,#253954,#253955,#253956,#253957,#253958,#253959,
#253960,#253961,#253962,#253963,#253964,#253965,#253966,#253967,#253968,
#253969,#253970,#253971,#253972,#253973,#253974,#253975,#253976,#253977,
#253978,#253979,#253980,#253981,#253982,#253983,#253984,#253985,#253986,
#253987,#253988,#253989,#253990,#253991),.UNSPECIFIED.,.F.,.F.,(4,3,3,3,
3,3,3,3,3,3,3,3,3,3,3,3,3,3,4),(0.000110053346854152,0.000527311722902683,
0.000718200211016838,0.000854122275951347,0.00126501374420219,0.00132634707517952,
0.0016865106123519,0.00193449393934221,0.00222985612782565,0.00251426340799237,
0.0025426408035049,0.00300412786903708,0.00333765384253382,0.00375893453183027,
0.00409210357719504,0.00415888746486192,0.00449321052529251,0.00480933253544403,
0.00497522826015564),.UNSPECIFIED.);
#5232=B_SPLINE_CURVE_WITH_KNOTS('',3,(#253995,#253996,#253997,#253998,#253999,
#254000,#254001,#254002,#254003,#254004,#254005,#254006,#254007,#254008,
#254009,#254010,#254011,#254012,#254013,#254014,#254015,#254016,#254017,
#254018,#254019,#254020,#254021,#254022,#254023,#254024,#254025,#254026,
#254027,#254028,#254029,#254030,#254031,#254032,#254033,#254034,#254035,
#254036,#254037,#254038,#254039,#254040,#254041,#254042,#254043),
 .UNSPECIFIED.,.F.,.F.,(4,3,3,3,3,3,3,3,3,3,3,3,3,3,3,3,4),(0.,0.000552804620541596,
0.000807500349756771,0.00120596662173938,0.00162007673419107,0.00218647027691998,
0.00241193324347875,0.0024321931256513,0.00283904062399194,0.00315006133501802,
0.0032484770180609,0.00361789986521813,0.00391885772790124,0.00407541417391128,
0.00422088317608781,0.00461166893077222,0.00482386648695749),
 .UNSPECIFIED.);
#5233=B_SPLINE_CURVE_WITH_KNOTS('',3,(#254045,#254046,#254047,#254048),
 .UNSPECIFIED.,.F.,.F.,(4,4),(9.81307786677359E-18,0.000614424279130633),
 .UNSPECIFIED.);
#5234=B_SPLINE_CURVE_WITH_KNOTS('',3,(#254052,#254053,#254054,#254055),
 .UNSPECIFIED.,.F.,.F.,(4,4),(-1.43540833570327E-5,0.000600070195786076),
 .UNSPECIFIED.);
#5235=B_SPLINE_CURVE_WITH_KNOTS('',3,(#254057,#254058,#254059,#254060,#254061,
#254062,#254063,#254064,#254065,#254066,#254067,#254068,#254069,#254070,
#254071,#254072,#254073,#254074,#254075,#254076,#254077,#254078,#254079,
#254080,#254081,#254082,#254083,#254084,#254085,#254086,#254087,#254088,
#254089,#254090,#254091,#254092,#254093,#254094,#254095,#254096,#254097,
#254098,#254099,#254100,#254101,#254102,#254103,#254104,#254105),
 .UNSPECIFIED.,.F.,.F.,(4,3,3,3,3,3,3,3,3,3,3,3,3,3,3,3,4),(0.000110053346854173,
0.000473524686504124,0.000718200211016846,0.000901529016375351,0.00127176706121883,
0.00132634707517952,0.00172429792281351,0.00193449393934219,0.00223976927323974,
0.00254238596260925,0.00254264080350487,0.00299415722452071,0.00335632568019801,
0.00375893453183022,0.00415022436231754,0.00456272631123656,0.00497522826015557),
 .UNSPECIFIED.);
#5236=B_SPLINE_CURVE_WITH_KNOTS('',3,(#254109,#254110,#254111,#254112,#254113,
#254114,#254115,#254116,#254117,#254118,#254119,#254120,#254121,#254122,
#254123,#254124,#254125,#254126,#254127,#254128,#254129,#254130,#254131,
#254132,#254133,#254134,#254135,#254136,#254137,#254138,#254139,#254140,
#254141,#254142,#254143,#254144,#254145,#254146,#254147,#254148,#254149,
#254150,#254151,#254152,#254153,#254154,#254155,#254156,#254157),
 .UNSPECIFIED.,.F.,.F.,(4,3,3,3,3,3,3,3,3,3,3,3,3,3,3,3,4),(0.,0.000552804620209682,
0.000807500349754742,0.00120596662173942,0.00162007673419038,0.00218647027609432,
0.00241193324347884,0.00243219312565006,0.00283904062398959,0.00315006133491644,
0.00324847701805861,0.00361789986521826,0.00391885772790331,0.00407541417390897,
0.00422088317608797,0.00461166893048689,0.00482386648695767),
 .UNSPECIFIED.);
#5237=B_SPLINE_CURVE_WITH_KNOTS('',3,(#254159,#254160,#254161,#254162),
 .UNSPECIFIED.,.F.,.F.,(4,4),(4.9065389333868E-18,0.000614424279130669),
 .UNSPECIFIED.);
#5238=B_SPLINE_CURVE_WITH_KNOTS('',3,(#254165,#254166,#254167,#254168,#254169,
#254170,#254171,#254172,#254173,#254174),.UNSPECIFIED.,.F.,.F.,(4,3,3,4),
(0.,0.00254000000002352,0.0127000000030823,0.0229583837181861),
 .UNSPECIFIED.);
#5239=B_SPLINE_CURVE_WITH_KNOTS('',3,(#254184,#254185,#254186,#254187,#254188,
#254189),.UNSPECIFIED.,.F.,.F.,(4,2,4),(-0.951075535059639,-0.475537767529819,
0.),.UNSPECIFIED.);
#5240=B_SPLINE_CURVE_WITH_KNOTS('',3,(#254197,#254198,#254199,#254200,#254201,
#254202,#254203,#254204,#254205,#254206,#254207,#254208,#254209,#254210,
#254211,#254212,#254213,#254214,#254215,#254216,#254217,#254218,#254219,
#254220,#254221,#254222,#254223,#254224,#254225,#254226,#254227,#254228,
#254229,#254230,#254231,#254232,#254233,#254234,#254235,#254236,#254237,
#254238,#254239,#254240,#254241,#254242,#254243,#254244,#254245,#254246,
#254247,#254248),.UNSPECIFIED.,.F.,.F.,(4,3,3,3,3,3,3,3,3,3,3,3,3,3,3,3,
3,4),(-3.16252941868488E-5,0.00137437432052449,0.00276766024128256,0.00349864849718784,
0.00351135631713655,0.00538023332270873,0.00702892228856252,0.00704872624461305,
0.00857771963899053,0.00879405918424988,0.00881347799615429,0.0105591960799372,
0.0105751229197932,0.0120513358719185,0.0123243329756246,0.0123340950401616,
0.0133922117480619,0.014089469871312),.UNSPECIFIED.);
#5241=B_SPLINE_CURVE_WITH_KNOTS('',3,(#254261,#254262,#254263,#254264,#254265,
#254266,#254267,#254268,#254269,#254270,#254271,#254272,#254273,#254274,
#254275,#254276,#254277,#254278,#254279,#254280,#254281,#254282,#254283,
#254284,#254285,#254286,#254287,#254288,#254289,#254290,#254291,#254292,
#254293,#254294,#254295,#254296,#254297,#254298,#254299,#254300,#254301,
#254302,#254303,#254304,#254305,#254306,#254307,#254308,#254309,#254310,
#254311,#254312,#254313,#254314,#254315,#254316,#254317,#254318),
 .UNSPECIFIED.,.F.,.F.,(4,3,3,3,3,3,3,3,3,3,3,3,3,3,3,3,3,3,3,4),(0.,0.00104968525641989,
0.001741380883755,0.00175109663942472,0.00321596412665287,0.00348633037654304,
0.00350219327884944,0.00523393136927482,0.00525328991827416,0.00677027115516066,
0.00698461442054001,0.00700438655769888,0.00885850868698763,0.0104937842336623,
0.0105065798365484,0.0115780826059013,0.0122576764759731,0.0131332247956855,
0.0135709989555417,0.0140087731153979),.UNSPECIFIED.);
#5242=B_SPLINE_CURVE_WITH_KNOTS('',3,(#254326,#254327,#254328,#254329,#254330,
#254331,#254332,#254333,#254334,#254335,#254336,#254337,#254338,#254339,
#254340,#254341,#254342,#254343,#254344,#254345,#254346,#254347,#254348,
#254349,#254350,#254351,#254352,#254353,#254354,#254355,#254356,#254357,
#254358,#254359,#254360,#254361,#254362,#254363,#254364,#254365,#254366,
#254367,#254368,#254369,#254370,#254371,#254372,#254373,#254374,#254375,
#254376,#254377),.UNSPECIFIED.,.F.,.F.,(4,3,3,3,3,3,3,3,3,3,3,3,3,3,3,3,
3,4),(-3.16252941869288E-5,0.00137437432795194,0.00276766023004491,0.00349864849718778,
0.0035113563171365,0.00538023332080317,0.00702892228856249,0.00704872624461302,
0.00857771966000481,0.00879405918424986,0.00881347799615426,0.0105591960799372,
0.0105751229197931,0.0120513358492157,0.0123243329756246,0.0123340950401616,
0.0133922117446449,0.014089469871312),.UNSPECIFIED.);
#5243=B_SPLINE_CURVE_WITH_KNOTS('',3,(#254406,#254407,#254408,#254409,#254410,
#254411,#254412,#254413,#254414,#254415,#254416,#254417,#254418,#254419,
#254420,#254421,#254422,#254423,#254424,#254425,#254426,#254427,#254428,
#254429,#254430,#254431,#254432,#254433,#254434,#254435,#254436,#254437,
#254438,#254439,#254440,#254441,#254442,#254443,#254444,#254445,#254446,
#254447,#254448,#254449,#254450,#254451,#254452,#254453,#254454,#254455,
#254456,#254457,#254458,#254459,#254460,#254461,#254462,#254463),
 .UNSPECIFIED.,.F.,.F.,(4,3,3,3,3,3,3,3,3,3,3,3,3,3,3,3,3,3,3,4),(0.,0.00104968525301761,
0.001741380883755,0.00175109663942474,0.00321596410406456,0.0034863303765431,
0.00350219327884948,0.00523393136927486,0.00525328991827421,0.00677027117601199,
0.00698461442054009,0.00700438655769895,0.0088585086860334,0.0104937842336624,
0.0105065798365484,0.0115780826096491,0.0122576764759731,0.0131332247956855,
0.0135709989555417,0.0140087731153978),.UNSPECIFIED.);
#5244=B_SPLINE_CURVE_WITH_KNOTS('',3,(#254466,#254467,#254468,#254469,#254470,
#254471,#254472,#254473,#254474,#254475,#254476,#254477,#254478,#254479,
#254480,#254481,#254482,#254483,#254484,#254485,#254486,#254487,#254488,
#254489,#254490,#254491,#254492,#254493,#254494,#254495,#254496,#254497,
#254498,#254499,#254500,#254501,#254502,#254503,#254504,#254505,#254506,
#254507,#254508,#254509,#254510,#254511,#254512,#254513,#254514,#254515,
#254516,#254517),.UNSPECIFIED.,.F.,.F.,(4,3,3,3,3,3,3,3,3,3,3,3,3,3,3,3,
3,4),(-3.16252941868488E-5,0.00137437432439234,0.0027676602298183,0.00349864849718784,
0.00351135631713652,0.00538023331410978,0.00702892228856252,0.00704872624461304,
0.00857771966078142,0.00879405918424988,0.00881347799615428,0.0105591960799372,
0.0105751229197931,0.012051335889654,0.0123243329756246,0.0123340950401616,
0.0133922117516399,0.014089469871312),.UNSPECIFIED.);
#5245=B_SPLINE_CURVE_WITH_KNOTS('',3,(#254526,#254527,#254528,#254529,#254530,
#254531,#254532,#254533,#254534,#254535,#254536,#254537,#254538,#254539,
#254540,#254541,#254542,#254543,#254544,#254545,#254546,#254547,#254548,
#254549,#254550,#254551,#254552,#254553,#254554,#254555,#254556,#254557,
#254558,#254559,#254560,#254561,#254562,#254563,#254564,#254565,#254566,
#254567,#254568,#254569,#254570,#254571,#254572,#254573,#254574,#254575,
#254576,#254577,#254578,#254579,#254580,#254581,#254582,#254583),
 .UNSPECIFIED.,.F.,.F.,(4,3,3,3,3,3,3,3,3,3,3,3,3,3,3,3,3,3,3,4),(0.,0.00104968525999275,
0.00174138088375498,0.00175109663942472,0.00321596414413303,0.00348633037654304,
0.00350219327884944,0.00523393136927485,0.00525328991827416,0.00677027117696927,
0.00698461442053999,0.00700438655769888,0.00885850867811475,0.0104937842336624,
0.0105065798365484,0.0115780826069947,0.0122576764759731,0.0131332247956855,
0.0135709989555417,0.0140087731153979),.UNSPECIFIED.);
#5246=B_SPLINE_CURVE_WITH_KNOTS('',3,(#254589,#254590,#254591,#254592,#254593,
#254594),.UNSPECIFIED.,.F.,.F.,(4,2,4),(-2.85874066322165,-2.38320289569183,
-1.907665128162),.UNSPECIFIED.);
#5247=B_SPLINE_CURVE_WITH_KNOTS('',3,(#254599,#254600,#254601,#254602,#254603,
#254604,#254605,#254606,#254607,#254608,#254609,#254610,#254611,#254612,
#254613,#254614,#254615,#254616,#254617,#254618,#254619,#254620,#254621,
#254622,#254623,#254624,#254625,#254626,#254627,#254628,#254629,#254630,
#254631,#254632,#254633,#254634,#254635,#254636,#254637,#254638,#254639,
#254640,#254641,#254642,#254643,#254644,#254645,#254646,#254647,#254648,
#254649,#254650,#254651,#254652,#254653,#254654,#254655,#254656),
 .UNSPECIFIED.,.F.,.F.,(4,3,3,3,3,3,3,3,3,3,3,3,3,3,3,3,3,3,3,4),(0.,0.00131752569946196,
0.00263505139892392,0.00439593787358465,0.00526189587671845,0.00527010279784784,
0.0105240963355105,0.0105402055956957,0.0170741315263014,0.0210484972404,
0.0210804111913913,0.0263355116903984,0.0315906121894055,0.031620616787087,
0.0336558605474688,0.0356821662679883,0.0368793854111903,0.0388917800756179,
0.0408753537649422,0.0421608223827827),.UNSPECIFIED.);
#5248=B_SPLINE_CURVE_WITH_KNOTS('',3,(#254710,#254711,#254712,#254713,#254714,
#254715,#254716,#254717,#254718,#254719,#254720,#254721,#254722,#254723,
#254724,#254725,#254726,#254727,#254728,#254729,#254730,#254731,#254732,
#254733,#254734,#254735,#254736,#254737,#254738,#254739,#254740,#254741,
#254742,#254743,#254744,#254745,#254746,#254747,#254748,#254749,#254750,
#254751,#254752,#254753,#254754,#254755),.UNSPECIFIED.,.F.,.F.,(4,3,3,3,
3,3,3,3,3,3,3,3,3,3,3,4),(0.,0.000232179668578841,0.000466221379334127,
0.00069011536363699,0.0010353712589054,0.00138023072727398,0.00207034609091097,
0.00276046145454796,0.00345057681818495,0.00414069218182194,0.00444163650088071,
0.00474476786788454,0.00483080754545894,0.00514271123354814,0.00545551728654251,
0.00552092290909593),.UNSPECIFIED.);
#5249=B_SPLINE_CURVE_WITH_KNOTS('',3,(#254762,#254763,#254764,#254765,#254766,
#254767,#254768,#254769,#254770,#254771,#254772,#254773,#254774,#254775,
#254776,#254777,#254778,#254779,#254780,#254781,#254782,#254783,#254784,
#254785,#254786,#254787,#254788,#254789,#254790,#254791,#254792,#254793,
#254794,#254795,#254796,#254797,#254798,#254799,#254800,#254801,#254802,
#254803,#254804,#254805,#254806,#254807),.UNSPECIFIED.,.F.,.F.,(4,3,3,3,
3,3,3,3,3,3,3,3,3,3,3,4),(0.,0.000235240533226937,0.000472127618779121,
0.00068965544306545,0.00103448316459817,0.0013793108861309,0.00206896632919635,
0.0027586217722618,0.00344827721532725,0.0041379326583927,0.00442075645279172,
0.0047045278060221,0.00482758810145815,0.00512139192932336,0.00541413800930076,
0.0055172435445236),.UNSPECIFIED.);
#5250=B_SPLINE_CURVE_WITH_KNOTS('',3,(#254811,#254812,#254813,#254814),
 .UNSPECIFIED.,.F.,.F.,(4,4),(0.,0.0224906085590336),.UNSPECIFIED.);
#5251=B_SPLINE_CURVE_WITH_KNOTS('',3,(#254820,#254821,#254822,#254823,#254824,
#254825,#254826,#254827,#254828,#254829),.UNSPECIFIED.,.F.,.F.,(4,2,2,2,
4),(-0.0398721478365828,-0.0302776007344581,-0.019948876411194,-0.0096621711043431,
-4.21224481406135E-8),.UNSPECIFIED.);
#5252=B_SPLINE_CURVE_WITH_KNOTS('',3,(#254831,#254832,#254833,#254834,#254835,
#254836,#254837),.UNSPECIFIED.,.F.,.F.,(4,3,4),(-0.000246059622236046,0.,
1.60099170077638E-5),.UNSPECIFIED.);
#5253=B_SPLINE_CURVE_WITH_KNOTS('',3,(#254839,#254840,#254841,#254842,#254843,
#254844),.UNSPECIFIED.,.F.,.F.,(4,2,4),(-0.0148199167117932,-0.00741824557827452,
-2.07859943751379E-6),.UNSPECIFIED.);
#5254=B_SPLINE_CURVE_WITH_KNOTS('',3,(#254855,#254856,#254857,#254858),
 .UNSPECIFIED.,.F.,.F.,(4,4),(0.00255945989202331,0.0250500684510569),
 .UNSPECIFIED.);
#5255=B_SPLINE_CURVE_WITH_KNOTS('',3,(#254864,#254865,#254866,#254867,#254868,
#254869),.UNSPECIFIED.,.F.,.F.,(4,2,4),(2.07859913676084E-6,0.00741824557851883,
0.014819916713439),.UNSPECIFIED.);
#5256=B_SPLINE_CURVE_WITH_KNOTS('',3,(#254871,#254872,#254873,#254874,#254875,
#254876,#254877),.UNSPECIFIED.,.F.,.F.,(4,3,4),(0.000666505089407319,0.000682515006394785,
0.000928574628629964),.UNSPECIFIED.);
#5257=B_SPLINE_CURVE_WITH_KNOTS('',3,(#254878,#254879,#254880,#254881,#254882,
#254883,#254884,#254885,#254886,#254887),.UNSPECIFIED.,.F.,.F.,(4,2,2,2,
4),(1.04282415750237E-8,0.00965213814703536,0.0199382545415243,0.030267394120979,
0.0398723888738878),.UNSPECIFIED.);
#5258=B_SPLINE_CURVE_WITH_KNOTS('',3,(#254890,#254891,#254892,#254893,#254894,
#254895,#254896,#254897,#254898,#254899,#254900,#254901,#254902,#254903,
#254904,#254905,#254906,#254907,#254908,#254909,#254910,#254911,#254912,
#254913,#254914,#254915,#254916,#254917),.UNSPECIFIED.,.F.,.F.,(4,3,3,3,
3,3,3,3,3,4),(1.77758317468082E-12,0.00346922799309708,0.00495442825517768,
0.00743164238276653,0.00888406179046178,0.00990885651035537,0.0124762492994206,
0.0150579051677044,0.0176593450599696,0.0198177130127836),.UNSPECIFIED.);
#5259=B_SPLINE_CURVE_WITH_KNOTS('',3,(#254926,#254927,#254928,#254929,#254930,
#254931,#254932,#254933,#254934,#254935,#254936,#254937,#254938,#254939,
#254940,#254941,#254942,#254943,#254944,#254945,#254946,#254947,#254948,
#254949,#254950,#254951,#254952,#254953,#254954,#254955,#254956,#254957,
#254958,#254959,#254960,#254961,#254962),.UNSPECIFIED.,.F.,.F.,(4,3,3,3,
3,3,3,3,3,3,3,3,4),(0.,0.00168691413199172,0.00335228412618897,0.00495034605026231,
0.00800843391090747,0.00989931177900222,0.00990069210052463,0.0123758651256558,
0.0124257497720468,0.0148510381507869,0.0149523121298537,0.0179692979973849,
0.0198013842010493),.UNSPECIFIED.);
#5260=B_SPLINE_CURVE_WITH_KNOTS('',3,(#254964,#254965,#254966,#254967,#254968,
#254969),.UNSPECIFIED.,.F.,.F.,(4,2,4),(5.82408502082562E-10,0.0170530403484513,
0.0341060806969008),.UNSPECIFIED.);
#5261=B_SPLINE_CURVE_WITH_KNOTS('',3,(#254971,#254972,#254973,#254974,#254975,
#254976,#254977,#254978,#254979,#254980,#254981,#254982,#254983,#254984,
#254985,#254986),.UNSPECIFIED.,.F.,.F.,(4,2,2,2,2,2,2,4),(0.000399405979664551,
0.00293135834355028,0.00546331070743601,0.0105272154352075,0.0206550248907504,
0.0307828343462933,0.0358467390740648,0.0409106438018362),.UNSPECIFIED.);
#5262=B_SPLINE_CURVE_WITH_KNOTS('',3,(#254987,#254988,#254989,#254990,#254991,
#254992),.UNSPECIFIED.,.F.,.F.,(4,2,4),(1.4304896245382E-17,0.0170530431506666,
0.0341060857189264),.UNSPECIFIED.);
#5263=B_SPLINE_CURVE_WITH_KNOTS('',3,(#255006,#255007,#255008,#255009,#255010,
#255011,#255012,#255013,#255014,#255015,#255016,#255017,#255018,#255019,
#255020,#255021),.UNSPECIFIED.,.F.,.F.,(4,3,3,3,3,4),(0.,0.0174001654419337,
0.0175045710703209,0.0261885013107201,0.0339450683097833,0.0348003308838674),
 .UNSPECIFIED.);
#5264=B_SPLINE_CURVE_WITH_KNOTS('',3,(#255031,#255032,#255033,#255034,#255035,
#255036,#255037,#255038,#255039,#255040,#255041,#255042,#255043),
 .UNSPECIFIED.,.F.,.F.,(4,3,3,3,4),(1.73472347597681E-18,0.00776408085901727,
0.0172957528190991,0.0174001584052762,0.0348003168105524),.UNSPECIFIED.);
#5265=B_SPLINE_CURVE_WITH_KNOTS('',3,(#255101,#255102,#255103,#255104,#255105,
#255106,#255107,#255108,#255109,#255110,#255111,#255112,#255113,#255114,
#255115,#255116,#255117,#255118,#255119,#255120,#255121,#255122,#255123,
#255124,#255125,#255126,#255127,#255128,#255129,#255130,#255131,#255132,
#255133,#255134,#255135,#255136,#255137,#255138,#255139,#255140,#255141,
#255142,#255143,#255144,#255145,#255146,#255147,#255148,#255149,#255150,
#255151,#255152),.UNSPECIFIED.,.F.,.F.,(4,3,3,3,3,3,3,3,3,3,3,3,3,3,3,3,
3,4),(-1.27903842355164E-5,0.,1.7463453400642E-5,3.50634018027296E-5,5.46656284338268E-5,
6.42421178660838E-5,6.64687762176374E-5,7.98821467223567E-5,9.02009949650424E-5,
9.32955172270761E-5,0.000100882589541566,0.000107962219828767,0.000114708247948279,
0.00011645022918071,0.000125670415610406,0.00013794360194898,0.000148213929951037,
0.000149858708640316),.UNSPECIFIED.);
#5266=B_SPLINE_CURVE_WITH_KNOTS('',3,(#255154,#255155,#255156,#255157,#255158,
#255159,#255160),.UNSPECIFIED.,.F.,.F.,(4,3,4),(0.000236530395619719,0.00031959462537318,
0.000330551443059626),.UNSPECIFIED.);
#5267=B_SPLINE_CURVE_WITH_KNOTS('',3,(#255166,#255167,#255168,#255169,#255170,
#255171,#255172),.UNSPECIFIED.,.F.,.F.,(4,3,4),(-1.00797019180758E-5,7.30168454413691E-5,
8.39413455213995E-5),.UNSPECIFIED.);
#5268=B_SPLINE_CURVE_WITH_KNOTS('',3,(#255174,#255175,#255176,#255177,#255178,
#255179,#255180,#255181,#255182,#255183,#255184,#255185,#255186,#255187,
#255188,#255189,#255190,#255191,#255192,#255193,#255194,#255195,#255196,
#255197,#255198,#255199,#255200,#255201,#255202,#255203,#255204,#255205,
#255206,#255207,#255208,#255209,#255210,#255211,#255212,#255213,#255214,
#255215,#255216,#255217,#255218,#255219,#255220,#255221,#255222),
 .UNSPECIFIED.,.F.,.F.,(4,3,3,3,3,3,3,3,3,3,3,3,3,3,3,3,4),(7.70239753203427E-14,
1.55924936070291E-5,2.35799864220384E-5,3.11849871370342E-5,3.5511652671198E-5,
4.31537913197463E-5,5.12752739862805E-5,5.54871328695572E-5,6.55863816260145E-5,
7.74044245036072E-5,7.80454628060054E-5,8.48409347506814E-5,0.000103972508418179,
0.000121518636800461,0.000138783636112226,0.00014916663373815,0.000161957017967162),
 .UNSPECIFIED.);
#5269=B_SPLINE_CURVE_WITH_KNOTS('',3,(#255226,#255227,#255228,#255229,#255230,
#255231,#255232,#255233,#255234,#255235,#255236,#255237,#255238,#255239,
#255240,#255241,#255242,#255243,#255244,#255245,#255246,#255247,#255248,
#255249,#255250,#255251,#255252,#255253,#255254,#255255,#255256,#255257,
#255258,#255259,#255260,#255261,#255262,#255263,#255264,#255265,#255266,
#255267,#255268,#255269,#255270,#255271,#255272,#255273,#255274,#255275,
#255276,#255277),.UNSPECIFIED.,.F.,.F.,(4,3,3,3,3,3,3,3,3,3,3,3,3,3,3,3,
3,4),(-1.27903842356209E-5,0.,1.74634534073477E-5,3.50634018159729E-5,5.46656284561953E-5,
6.42421178650527E-5,6.64687762176552E-5,7.98821467213225E-5,9.02009949648931E-5,
9.32955172249898E-5,0.000100882589539224,0.000107962219826057,0.000114708247945179,
0.000116450229181048,0.000125670415610166,0.000137943601951022,0.000148213929942978,
0.000149858708640884),.UNSPECIFIED.);
#5270=B_SPLINE_CURVE_WITH_KNOTS('',3,(#255279,#255280,#255281,#255282,#255283,
#255284,#255285),.UNSPECIFIED.,.F.,.F.,(4,3,4),(0.000236530395620193,0.000319594623033558,
0.000330551443059687),.UNSPECIFIED.);
#5271=B_SPLINE_CURVE_WITH_KNOTS('',3,(#255303,#255304,#255305,#255306,#255307,
#255308,#255309),.UNSPECIFIED.,.F.,.F.,(4,3,4),(-1.00797019179348E-5,7.30168513305268E-5,
8.39413455215476E-5),.UNSPECIFIED.);
#5272=B_SPLINE_CURVE_WITH_KNOTS('',3,(#255310,#255311,#255312,#255313,#255314,
#255315,#255316,#255317,#255318,#255319,#255320,#255321,#255322,#255323,
#255324,#255325,#255326,#255327,#255328,#255329,#255330,#255331,#255332,
#255333,#255334,#255335,#255336,#255337,#255338,#255339,#255340,#255341,
#255342,#255343,#255344,#255345,#255346,#255347,#255348,#255349,#255350,
#255351,#255352,#255353,#255354,#255355,#255356,#255357,#255358),
 .UNSPECIFIED.,.F.,.F.,(4,3,3,3,3,3,3,3,3,3,3,3,3,3,3,3,4),(7.6239948049063E-14,
1.55924936059415E-5,2.35799886190525E-5,3.1184987135643E-5,3.5511663807096E-5,
4.31538029420733E-5,5.12752864215393E-5,5.54871407305369E-5,6.5586390413675E-5,
7.7404434382236E-5,7.80454628009842E-5,8.4840940844391E-5,0.00010397251409257,
0.000121518642655327,0.000138783642360409,0.000149166633737892,0.000161957017966969),
 .UNSPECIFIED.);
#5273=B_SPLINE_CURVE_WITH_KNOTS('',3,(#255365,#255366,#255367,#255368,#255369,
#255370,#255371,#255372,#255373,#255374,#255375,#255376,#255377,#255378,
#255379,#255380,#255381,#255382,#255383,#255384,#255385,#255386,#255387,
#255388,#255389,#255390,#255391,#255392,#255393,#255394,#255395,#255396,
#255397,#255398,#255399,#255400,#255401,#255402,#255403,#255404,#255405,
#255406,#255407,#255408,#255409,#255410,#255411,#255412,#255413,#255414,
#255415,#255416),.UNSPECIFIED.,.F.,.F.,(4,3,3,3,3,3,3,3,3,3,3,3,3,3,3,3,
3,4),(-1.27903842354479E-5,0.,1.74634534010109E-5,3.50634018038132E-5,5.46656284408684E-5,
6.42421178641914E-5,6.64687762172822E-5,7.98821467208371E-5,9.02009949633172E-5,
9.32955172243919E-5,0.000100882589539266,0.000107962219826603,0.000114708247946188,
0.000116450229181059,0.000125670415611108,0.000137943601956876,0.000148213929940526,
0.000149858708640885),.UNSPECIFIED.);
#5274=B_SPLINE_CURVE_WITH_KNOTS('',3,(#255418,#255419,#255420,#255421,#255422,
#255423,#255424),.UNSPECIFIED.,.F.,.F.,(4,3,4),(0.000236530395620128,0.000319594622622922,
0.000330551443059518),.UNSPECIFIED.);
#5275=B_SPLINE_CURVE_WITH_KNOTS('',3,(#255448,#255449,#255450,#255451,#255452,
#255453,#255454),.UNSPECIFIED.,.F.,.F.,(4,3,4),(-1.00797019178162E-5,7.30168515357015E-5,
8.3941345521282E-5),.UNSPECIFIED.);
#5276=B_SPLINE_CURVE_WITH_KNOTS('',3,(#255456,#255457,#255458,#255459,#255460,
#255461,#255462,#255463,#255464,#255465,#255466,#255467,#255468,#255469,
#255470,#255471,#255472,#255473,#255474,#255475,#255476,#255477,#255478,
#255479,#255480,#255481,#255482,#255483,#255484,#255485,#255486,#255487,
#255488,#255489,#255490,#255491,#255492,#255493,#255494,#255495,#255496,
#255497,#255498,#255499,#255500,#255501,#255502,#255503,#255504),
 .UNSPECIFIED.,.F.,.F.,(4,3,3,3,3,3,3,3,3,3,3,3,3,3,3,3,4),(6.92532125292866E-14,
1.55924936024845E-5,2.35799888310557E-5,3.11849871357157E-5,3.55116648883676E-5,
4.31538040729246E-5,5.12752876341333E-5,5.54871414935716E-5,6.55863912699049E-5,
7.74044353491455E-5,7.80454628014266E-5,8.48409414355659E-5,0.000103972514645705,
0.00012151864322897,0.000138783642975998,0.000149166633737459,0.000161957017966677),
 .UNSPECIFIED.);
#5277=B_SPLINE_CURVE_WITH_KNOTS('',3,(#255512,#255513,#255514,#255515,#255516,
#255517,#255518,#255519,#255520,#255521,#255522,#255523,#255524,#255525,
#255526,#255527,#255528,#255529,#255530,#255531,#255532,#255533,#255534,
#255535,#255536,#255537,#255538,#255539,#255540,#255541,#255542,#255543,
#255544,#255545,#255546,#255547,#255548,#255549,#255550,#255551,#255552,
#255553,#255554,#255555,#255556,#255557,#255558,#255559,#255560,#255561,
#255562,#255563),.UNSPECIFIED.,.F.,.F.,(4,3,3,3,3,3,3,3,3,3,3,3,3,3,3,3,
3,4),(-1.27903842354613E-5,0.,1.746345340453E-5,3.50634018098178E-5,5.46656284383532E-5,
6.42421178639721E-5,6.64687762142466E-5,7.98821467187808E-5,9.02009949657256E-5,
9.32955172233151E-5,0.000100882589538758,0.000107962219826646,0.000114708247946761,
0.00011645022918108,0.00012567041561163,0.000137943601961324,0.000148213929933755,
0.000149858708641606),.UNSPECIFIED.);
#5278=B_SPLINE_CURVE_WITH_KNOTS('',3,(#255565,#255566,#255567,#255568,#255569,
#255570,#255571),.UNSPECIFIED.,.F.,.F.,(4,3,4),(0.000236530395619718,0.000319594617376154,
0.000330551443059305),.UNSPECIFIED.);
#5279=B_SPLINE_CURVE_WITH_KNOTS('',3,(#255596,#255597,#255598,#255599),
 .UNSPECIFIED.,.F.,.F.,(4,4),(1.04083408558608E-17,0.000776824705292365),
 .UNSPECIFIED.);
#5280=B_SPLINE_CURVE_WITH_KNOTS('',3,(#255602,#255603,#255604,#255605),
 .UNSPECIFIED.,.F.,.F.,(4,4),(0.,0.000776824705292377),.UNSPECIFIED.);
#5281=B_SPLINE_CURVE_WITH_KNOTS('',3,(#255607,#255608,#255609,#255610),
 .UNSPECIFIED.,.F.,.F.,(4,4),(3.46944695195361E-18,0.000776824705292372),
 .UNSPECIFIED.);
#5282=B_SPLINE_CURVE_WITH_KNOTS('',3,(#255611,#255612,#255613,#255614),
 .UNSPECIFIED.,.F.,.F.,(4,4),(0.,0.000776824705292378),.UNSPECIFIED.);
#5283=B_SPLINE_CURVE_WITH_KNOTS('',3,(#255616,#255617,#255618,#255619),
 .UNSPECIFIED.,.F.,.F.,(4,4),(3.46944695195361E-18,0.000776824705292372),
 .UNSPECIFIED.);
#5284=B_SPLINE_CURVE_WITH_KNOTS('',3,(#255620,#255621,#255622,#255623),
 .UNSPECIFIED.,.F.,.F.,(4,4),(0.,0.00077682470529238),.UNSPECIFIED.);
#5285=B_SPLINE_CURVE_WITH_KNOTS('',3,(#255627,#255628,#255629,#255630,#255631,
#255632,#255633,#255634,#255635,#255636,#255637,#255638,#255639,#255640,
#255641,#255642,#255643,#255644,#255645,#255646,#255647,#255648,#255649,
#255650,#255651,#255652,#255653,#255654,#255655,#255656,#255657,#255658,
#255659,#255660,#255661,#255662,#255663,#255664,#255665,#255666,#255667,
#255668,#255669,#255670,#255671,#255672,#255673,#255674,#255675,#255676,
#255677,#255678,#255679,#255680,#255681,#255682,#255683,#255684,#255685,
#255686,#255687,#255688,#255689,#255690,#255691,#255692,#255693),
 .UNSPECIFIED.,.F.,.F.,(4,3,3,3,3,3,3,3,3,3,3,3,3,3,3,3,3,3,3,3,3,3,4),
(4.9065389333868E-18,0.000187317538506277,0.000370529360731883,0.000549649653517671,
0.000585186929066945,0.000747835352058225,0.00090905754882324,0.00106903584072748,
0.00117037385813389,0.00139504516879083,0.00161858460257625,0.00175556078720083,
0.00198345805102534,0.0020481542517343,0.00213117924281626,0.00219445098400102,
0.00221273807553437,0.00222891957305618,0.00223102516706771,0.00226084972327193,
0.0022675993501344,0.00232401155250101,0.00234074771626781),
 .UNSPECIFIED.);
#5286=B_SPLINE_CURVE_WITH_KNOTS('',3,(#255708,#255709,#255710,#255711,#255712,
#255713,#255714),.UNSPECIFIED.,.F.,.F.,(4,3,4),(-1.6148217724202E-5,0.000301256797926397,
0.000615737100014097),.UNSPECIFIED.);
#5287=B_SPLINE_CURVE_WITH_KNOTS('',3,(#255715,#255716,#255717,#255718),
 .UNSPECIFIED.,.F.,.F.,(4,4),(0.,0.000264303642305848),.UNSPECIFIED.);
#5288=B_SPLINE_CURVE_WITH_KNOTS('',3,(#255721,#255722,#255723,#255724,#255725,
#255726,#255727,#255728,#255729,#255730,#255731,#255732,#255733,#255734,
#255735,#255736,#255737,#255738,#255739,#255740,#255741,#255742,#255743,
#255744,#255745,#255746,#255747,#255748,#255749,#255750,#255751,#255752,
#255753,#255754,#255755,#255756,#255757,#255758,#255759,#255760,#255761,
#255762,#255763,#255764,#255765,#255766,#255767,#255768,#255769,#255770,
#255771,#255772,#255773,#255774,#255775,#255776,#255777,#255778,#255779,
#255780,#255781,#255782,#255783,#255784,#255785,#255786,#255787),
 .UNSPECIFIED.,.F.,.F.,(4,3,3,3,3,3,3,3,3,3,3,3,3,3,3,3,3,3,3,3,3,3,4),
(1.98780968783202E-9,5.73414915694073E-5,7.42300839654611E-5,0.000104673148245408,
0.000111344132043346,0.000127856077372199,0.00012990115608229,0.000148458180121234,
0.00023314346664102,0.000296914372432783,0.000529593879008388,0.000593826757055878,
0.000836090912058093,0.00108017083919709,0.00118765152630205,0.00135313333384191,
0.00151932196905603,0.00168746877222913,0.00178147629554822,0.00194158715598329,
0.00210403684094403,0.00227214417361886,0.00237530106479439),
 .UNSPECIFIED.);
#5289=B_SPLINE_CURVE_WITH_KNOTS('',3,(#255803,#255804,#255805,#255806),
 .UNSPECIFIED.,.F.,.F.,(4,4),(7.2194514417634E-17,0.000264303642294797),
 .UNSPECIFIED.);
#5290=B_SPLINE_CURVE_WITH_KNOTS('',3,(#255807,#255808,#255809,#255810,#255811,
#255812,#255813),.UNSPECIFIED.,.F.,.F.,(4,3,4),(3.46944695195361E-18,0.000317405080301234,
0.000631885317751415),.UNSPECIFIED.);
#5291=B_SPLINE_CURVE_WITH_KNOTS('',3,(#255817,#255818,#255819,#255820,#255821,
#255822,#255823,#255824,#255825,#255826,#255827,#255828,#255829,#255830,
#255831,#255832,#255833,#255834,#255835,#255836,#255837,#255838,#255839,
#255840,#255841,#255842,#255843,#255844,#255845,#255846,#255847,#255848,
#255849,#255850,#255851,#255852,#255853,#255854,#255855,#255856,#255857,
#255858,#255859,#255860,#255861,#255862,#255863,#255864,#255865,#255866,
#255867,#255868,#255869,#255870,#255871,#255872,#255873,#255874,#255875,
#255876,#255877,#255878,#255879,#255880,#255881,#255882,#255883),
 .UNSPECIFIED.,.F.,.F.,(4,3,3,3,3,3,3,3,3,3,3,3,3,3,3,3,3,3,3,3,3,3,4),
(4.23499971748596E-17,0.000187317538506265,0.000370529360731306,0.000549649653516587,
0.000585186929067176,0.000747835352058548,0.000909057548823778,0.00106903584072817,
0.00117037385813431,0.00139504516879073,0.00161858460257628,0.00175556078720144,
0.00198345805102,0.002048154251735,0.00213117924281676,0.00219445098400178,
0.00221273807553513,0.00222891957305701,0.00223102516706848,0.00226084972327255,
0.00226759935013518,0.00232401155250177,0.00234074771626859),
 .UNSPECIFIED.);
#5292=B_SPLINE_CURVE_WITH_KNOTS('',3,(#255897,#255898,#255899,#255900,#255901,
#255902,#255903),.UNSPECIFIED.,.F.,.F.,(4,3,4),(-1.61482177233483E-5,0.000301256721641648,
0.000615737100014892),.UNSPECIFIED.);
#5293=B_SPLINE_CURVE_WITH_KNOTS('',3,(#255904,#255905,#255906,#255907),
 .UNSPECIFIED.,.F.,.F.,(4,4),(0.,0.000264303642305846),.UNSPECIFIED.);
#5294=B_SPLINE_CURVE_WITH_KNOTS('',3,(#255910,#255911,#255912,#255913,#255914,
#255915,#255916,#255917,#255918,#255919),.UNSPECIFIED.,.F.,.F.,(4,3,3,4),
(-3.83013078967852E-5,0.,0.000144401167384903,0.000501272209488935),
 .UNSPECIFIED.);
#5295=B_SPLINE_CURVE_WITH_KNOTS('',3,(#255921,#255922,#255923,#255924,#255925,
#255926,#255927,#255928,#255929,#255930,#255931,#255932,#255933,#255934,
#255935,#255936,#255937,#255938,#255939,#255940),.UNSPECIFIED.,.F.,.F.,
(4,2,2,2,2,2,2,2,2,4),(4.7385767894594E-6,2.26507325412358E-5,4.05628882930122E-5,
7.63871997965703E-5,0.000148035822803692,0.000291333068817939,0.000577927560846451,
0.00115111654490347,0.00172430552896048,0.0022974945130175),
 .UNSPECIFIED.);
#5296=B_SPLINE_CURVE_WITH_KNOTS('',3,(#255955,#255956,#255957,#255958),
 .UNSPECIFIED.,.F.,.F.,(4,4),(0.,0.00026430364229488),.UNSPECIFIED.);
#5297=B_SPLINE_CURVE_WITH_KNOTS('',3,(#255959,#255960,#255961,#255962,#255963,
#255964,#255965),.UNSPECIFIED.,.F.,.F.,(4,3,4),(3.46944695195361E-18,0.000317404992696139,
0.000631885317751336),.UNSPECIFIED.);
#5298=B_SPLINE_CURVE_WITH_KNOTS('',3,(#255969,#255970,#255971,#255972,#255973,
#255974,#255975,#255976,#255977,#255978,#255979,#255980,#255981,#255982,
#255983,#255984,#255985,#255986,#255987,#255988,#255989,#255990,#255991,
#255992,#255993,#255994,#255995,#255996,#255997,#255998,#255999,#256000,
#256001,#256002,#256003,#256004,#256005,#256006,#256007,#256008,#256009,
#256010,#256011,#256012,#256013,#256014,#256015,#256016,#256017,#256018,
#256019,#256020,#256021,#256022,#256023,#256024,#256025,#256026,#256027,
#256028,#256029,#256030,#256031,#256032,#256033,#256034,#256035),
 .UNSPECIFIED.,.F.,.F.,(4,3,3,3,3,3,3,3,3,3,3,3,3,3,3,3,3,3,3,3,3,3,4),
(0.,0.000187317538506216,0.000370529360731649,0.000549649653517311,0.000585186929066575,
0.000747835352057596,0.000909057548822561,0.00106903584072672,0.00117037385813315,
0.00139504516878895,0.00161858460257515,0.00175556078719972,0.00198345805101906,
0.00204815425173301,0.00213117924281621,0.00219445098399965,0.00221273807553298,
0.00222891957305496,0.00223102516706631,0.00226084972326921,0.00226759935013298,
0.00232401155249693,0.0023407477162663),.UNSPECIFIED.);
#5299=B_SPLINE_CURVE_WITH_KNOTS('',3,(#256049,#256050,#256051,#256052,#256053,
#256054,#256055),.UNSPECIFIED.,.F.,.F.,(4,3,4),(-1.61482177236942E-5,0.000301257027968063,
0.000615737100014811),.UNSPECIFIED.);
#5300=B_SPLINE_CURVE_WITH_KNOTS('',3,(#256056,#256057,#256058,#256059),
 .UNSPECIFIED.,.F.,.F.,(4,4),(0.,0.000264303642305761),.UNSPECIFIED.);
#5301=B_SPLINE_CURVE_WITH_KNOTS('',3,(#256062,#256063,#256064,#256065,#256066,
#256067,#256068,#256069,#256070,#256071,#256072,#256073,#256074,#256075,
#256076,#256077,#256078,#256079,#256080,#256081,#256082,#256083,#256084,
#256085,#256086,#256087,#256088,#256089,#256090,#256091,#256092,#256093,
#256094,#256095,#256096,#256097,#256098,#256099,#256100,#256101,#256102,
#256103,#256104,#256105,#256106,#256107,#256108,#256109,#256110,#256111,
#256112,#256113,#256114,#256115,#256116,#256117,#256118,#256119,#256120,
#256121,#256122,#256123,#256124,#256125,#256126,#256127,#256128),
 .UNSPECIFIED.,.F.,.F.,(4,3,3,3,3,3,3,3,3,3,3,3,3,3,3,3,3,3,3,3,3,3,4),
(1.98061349608262E-9,5.73415218899911E-5,7.4230076566389E-5,0.000104673137737296,
0.000111344124542838,0.000127856070079246,0.000129901148531068,0.000148458172519298,
0.00023314347760765,0.000296914364425009,0.000529593869959597,0.000593826748236463,
0.00083609090671776,0.00108017083758895,0.00118765151585936,0.00135313332319783,
0.00151932195821436,0.00168746876119618,0.00178147628348225,0.00194158714386398,
0.00210403682877481,0.00227214416139509,0.00237530105110514),
 .UNSPECIFIED.);
#5302=B_SPLINE_CURVE_WITH_KNOTS('',3,(#256143,#256144,#256145,#256146),
 .UNSPECIFIED.,.F.,.F.,(4,4),(1.2509268882771E-17,0.000264303642294947),
 .UNSPECIFIED.);
#5303=B_SPLINE_CURVE_WITH_KNOTS('',3,(#256147,#256148,#256149,#256150,#256151,
#256152,#256153),.UNSPECIFIED.,.F.,.F.,(4,3,4),(0.,0.000317405083030208,
0.000631885317751385),.UNSPECIFIED.);
#5304=B_SPLINE_CURVE_WITH_KNOTS('',3,(#256167,#256168,#256169,#256170),
 .UNSPECIFIED.,.F.,.F.,(4,4),(0.,0.00026430364229487),.UNSPECIFIED.);
#5305=B_SPLINE_CURVE_WITH_KNOTS('',3,(#256171,#256172,#256173,#256174,#256175,
#256176,#256177),.UNSPECIFIED.,.F.,.F.,(4,3,4),(3.46944695195361E-18,0.000317405268168359,
0.000631885317751483),.UNSPECIFIED.);
#5306=B_SPLINE_CURVE_WITH_KNOTS('',3,(#256191,#256192,#256193,#256194,#256195,
#256196,#256197),.UNSPECIFIED.,.F.,.F.,(4,3,4),(-1.61482177234426E-5,0.000301256699244678,
0.000615737100014854),.UNSPECIFIED.);
#5307=B_SPLINE_CURVE_WITH_KNOTS('',3,(#256198,#256199,#256200,#256201),
 .UNSPECIFIED.,.F.,.F.,(4,4),(0.,0.000264303642305819),.UNSPECIFIED.);
#5308=B_SPLINE_CURVE_WITH_KNOTS('',3,(#256271,#256272,#256273,#256274,#256275,
#256276,#256277,#256278,#256279,#256280,#256281,#256282,#256283,#256284,
#256285,#256286,#256287,#256288,#256289,#256290,#256291,#256292,#256293,
#256294,#256295,#256296,#256297,#256298,#256299,#256300,#256301,#256302,
#256303,#256304,#256305,#256306,#256307,#256308,#256309,#256310,#256311,
#256312,#256313,#256314,#256315,#256316,#256317,#256318,#256319),
 .UNSPECIFIED.,.F.,.F.,(4,3,3,3,3,3,3,3,3,3,3,3,3,3,3,3,4),(-3.28957225289004E-5,
0.00123839561282373,0.00246284557240642,0.00350220228306729,0.00356136795860099,
0.00529933412363224,0.00703730028866348,0.00712550648875341,0.0081204335483374,
0.00890034485054549,0.00977320546531314,0.0105723982942597,0.0106614349564065,
0.0118079342051501,0.0123965937508694,0.0134149359774125,0.0141074962998559),
 .UNSPECIFIED.);
#5309=B_SPLINE_CURVE_WITH_KNOTS('',3,(#256323,#256324,#256325,#256326,#256327,
#256328,#256329,#256330,#256331,#256332,#256333,#256334,#256335,#256336,
#256337,#256338,#256339,#256340,#256341,#256342,#256343,#256344,#256345,
#256346,#256347,#256348,#256349,#256350,#256351,#256352,#256353,#256354,
#256355,#256356,#256357,#256358,#256359,#256360,#256361,#256362,#256363,
#256364,#256365,#256366,#256367,#256368,#256369,#256370,#256371),
 .UNSPECIFIED.,.F.,.F.,(4,3,3,3,3,3,3,3,3,3,3,3,3,3,3,3,4),(-3.28957225289004E-5,
0.00123839561282583,0.00246284557240834,0.00350220228306729,0.00356136795860099,
0.00529933412363224,0.00703730028866348,0.00712550648875342,0.00812043354833833,
0.00890034485054549,0.00977320546531023,0.0105723982942597,0.0106614349564065,
0.0118079342051527,0.0123965937508694,0.0134149359774119,0.0141074962998559),
 .UNSPECIFIED.);
#5310=B_SPLINE_CURVE_WITH_KNOTS('',3,(#256462,#256463,#256464,#256465,#256466,
#256467,#256468,#256469,#256470,#256471,#256472,#256473,#256474,#256475,
#256476,#256477,#256478,#256479,#256480,#256481,#256482,#256483,#256484,
#256485,#256486,#256487,#256488,#256489,#256490,#256491,#256492,#256493,
#256494,#256495,#256496,#256497,#256498,#256499,#256500,#256501,#256502,
#256503,#256504,#256505,#256506,#256507,#256508,#256509,#256510),
 .UNSPECIFIED.,.F.,.F.,(4,3,3,3,3,3,3,3,3,3,3,3,3,3,3,3,4),(-3.28957225289672E-5,
0.00123839562134457,0.0024628455650959,0.00350220228306722,0.00356136795860092,
0.00529933412363217,0.00703730028866341,0.00712550648875332,0.00812043354890156,
0.00890034485054153,0.00977320546595051,0.0105723982942596,0.0106614349564063,
0.0118079342061304,0.0123965937508664,0.0134149359795621,0.0141074962998558),
 .UNSPECIFIED.);
#5311=B_SPLINE_CURVE_WITH_KNOTS('',3,(#256514,#256515,#256516,#256517,#256518,
#256519,#256520,#256521,#256522,#256523,#256524,#256525,#256526,#256527,
#256528,#256529,#256530,#256531,#256532,#256533,#256534,#256535,#256536,
#256537,#256538,#256539,#256540,#256541,#256542,#256543,#256544,#256545,
#256546,#256547,#256548,#256549,#256550,#256551,#256552,#256553,#256554,
#256555,#256556,#256557,#256558,#256559,#256560,#256561,#256562),
 .UNSPECIFIED.,.F.,.F.,(4,3,3,3,3,3,3,3,3,3,3,3,3,3,3,3,4),(-3.28957225289672E-5,
0.0012383956213515,0.00246284556510125,0.00350220228306722,0.00356136795860093,
0.00529933412363217,0.00703730028866341,0.00712550648875329,0.00812043354890009,
0.0089003448505415,0.00977320546595016,0.0105723982942596,0.0106614349564063,
0.01180793420613,0.0123965937508664,0.0134149359795605,0.0141074962998558),
 .UNSPECIFIED.);
#5312=B_SPLINE_CURVE_WITH_KNOTS('',3,(#256654,#256655,#256656,#256657,#256658,
#256659,#256660,#256661,#256662,#256663,#256664,#256665,#256666,#256667,
#256668,#256669,#256670,#256671,#256672,#256673,#256674,#256675,#256676,
#256677,#256678,#256679,#256680,#256681,#256682,#256683,#256684,#256685,
#256686,#256687,#256688,#256689,#256690,#256691,#256692,#256693,#256694,
#256695,#256696,#256697,#256698,#256699,#256700,#256701,#256702),
 .UNSPECIFIED.,.F.,.F.,(4,3,3,3,3,3,3,3,3,3,3,3,3,3,3,3,4),(-3.28957225289672E-5,
0.00123839562262854,0.00246284556740731,0.00350220228306722,0.0035613679586009,
0.00529933412363216,0.00703730028866341,0.00712550648875328,0.00812043354869755,
0.00890034485054217,0.00977320546566178,0.0105723982942596,0.0106614349564064,
0.0118079342049588,0.0123965937508674,0.0134149359781372,0.0141074962998558),
 .UNSPECIFIED.);
#5313=B_SPLINE_CURVE_WITH_KNOTS('',3,(#256706,#256707,#256708,#256709,#256710,
#256711,#256712,#256713,#256714,#256715,#256716,#256717,#256718,#256719,
#256720,#256721,#256722,#256723,#256724,#256725,#256726,#256727,#256728,
#256729,#256730,#256731,#256732,#256733,#256734,#256735,#256736,#256737,
#256738,#256739,#256740,#256741,#256742,#256743,#256744,#256745,#256746,
#256747,#256748,#256749,#256750,#256751,#256752,#256753,#256754),
 .UNSPECIFIED.,.F.,.F.,(4,3,3,3,3,3,3,3,3,3,3,3,3,3,3,3,4),(-3.28957225289672E-5,
0.00123839562262829,0.00246284556740624,0.00350220228306722,0.00356136795860091,
0.00529933412363216,0.00703730028866341,0.0071255064887533,0.00812043354869597,
0.00890034485054217,0.00977320546566605,0.0105723982942596,0.0106614349564064,
0.0118079342049593,0.0123965937508674,0.0134149359781345,0.0141074962998558),
 .UNSPECIFIED.);
#5314=B_SPLINE_CURVE_WITH_KNOTS('',3,(#256848,#256849,#256850,#256851,#256852,
#256853,#256854,#256855,#256856,#256857,#256858,#256859,#256860,#256861,
#256862,#256863,#256864,#256865,#256866,#256867,#256868,#256869,#256870,
#256871,#256872,#256873,#256874,#256875,#256876,#256877,#256878,#256879,
#256880,#256881,#256882,#256883,#256884,#256885,#256886,#256887,#256888,
#256889,#256890,#256891,#256892,#256893,#256894,#256895,#256896,#256897,
#256898,#256899,#256900,#256901,#256902,#256903,#256904,#256905,#256906,
#256907,#256908,#256909,#256910,#256911,#256912,#256913,#256914,#256915,
#256916,#256917,#256918,#256919,#256920,#256921,#256922,#256923,#256924,
#256925,#256926,#256927,#256928,#256929,#256930,#256931,#256932,#256933,
#256934,#256935,#256936,#256937,#256938,#256939,#256940,#256941,#256942,
#256943,#256944,#256945,#256946,#256947),.UNSPECIFIED.,.F.,.F.,(4,3,3,3,
3,3,3,3,3,3,3,3,3,3,3,3,3,3,3,3,3,3,3,3,3,3,3,3,3,3,3,3,3,4),(1.42043634129218E-9,
8.96508234963807E-5,0.000177139225359939,0.000196453687302178,0.000222064227861235,
0.000285479098213833,0.000349005642415524,0.000361856879033328,0.000392907374604338,
0.000507356384677131,0.000595775533469028,0.000684346942788586,0.000773468971709804,
0.000785814749208658,0.000832772345389435,0.000952902380893138,0.00107741065969588,
0.00117872212381298,0.00121565072790586,0.00131178235002056,0.00141569811404612,
0.00142936137630885,0.00155931596577564,0.0015716294984173,0.00165375706712277,
0.00184401976952065,0.00204137976398503,0.0021285000374069,0.00230460243506521,
0.00235744424762594,0.00259423468405583,0.00263013820146309,0.00296211475305905,
0.00314325899683457),.UNSPECIFIED.);
#5315=B_SPLINE_CURVE_WITH_KNOTS('',3,(#256952,#256953,#256954,#256955,#256956,
#256957,#256958,#256959,#256960,#256961,#256962,#256963,#256964,#256965,
#256966,#256967,#256968,#256969,#256970,#256971,#256972,#256973,#256974,
#256975,#256976,#256977,#256978,#256979,#256980,#256981,#256982,#256983,
#256984,#256985,#256986,#256987,#256988,#256989,#256990,#256991,#256992,
#256993,#256994,#256995,#256996,#256997,#256998,#256999,#257000,#257001,
#257002,#257003,#257004,#257005,#257006,#257007,#257008,#257009,#257010,
#257011,#257012,#257013,#257014,#257015,#257016,#257017,#257018,#257019,
#257020,#257021,#257022,#257023,#257024,#257025,#257026,#257027,#257028,
#257029,#257030,#257031,#257032,#257033,#257034,#257035,#257036,#257037,
#257038,#257039,#257040,#257041,#257042,#257043,#257044,#257045,#257046,
#257047,#257048,#257049,#257050,#257051),.UNSPECIFIED.,.F.,.F.,(4,3,3,3,
3,3,3,3,3,3,3,3,3,3,3,3,3,3,3,3,3,3,3,3,3,3,3,3,3,3,3,3,3,4),(6.93889390390723E-18,
0.000232066433642932,0.000444177580050074,0.000518385099123644,0.000734102786663995,
0.00079015638993006,0.000993487732790287,0.00102299023054961,0.00119225943856918,
0.00134764700037811,0.00150263588856933,0.00158031277986011,0.00171536369190904,
0.00184243086348886,0.00194346242503313,0.00197539097482514,0.00208159421176549,
0.00218487525328951,0.00228393672716245,0.0023319957435332,0.00237046916979017,
0.00246124899505445,0.00255227503608586,0.00264431970448832,0.00265740253517428,
0.0027655473647552,0.00280202928405062,0.00287180839700997,0.00294158750996931,
0.00296308646223771,0.00302593425586122,0.00308943159919426,0.00315434926414339,
0.00316062418320347),.UNSPECIFIED.);
#5316=B_SPLINE_CURVE_WITH_KNOTS('',3,(#257053,#257054,#257055,#257056,#257057,
#257058,#257059,#257060,#257061,#257062,#257063,#257064,#257065,#257066,
#257067,#257068,#257069,#257070,#257071,#257072,#257073,#257074,#257075,
#257076,#257077,#257078,#257079,#257080,#257081,#257082,#257083,#257084,
#257085,#257086,#257087,#257088,#257089,#257090,#257091,#257092,#257093,
#257094,#257095,#257096,#257097,#257098,#257099,#257100,#257101,#257102,
#257103,#257104,#257105,#257106,#257107,#257108,#257109,#257110,#257111,
#257112,#257113,#257114,#257115,#257116,#257117,#257118,#257119,#257120,
#257121,#257122,#257123,#257124,#257125,#257126,#257127,#257128,#257129,
#257130,#257131,#257132,#257133,#257134,#257135,#257136,#257137,#257138,
#257139,#257140,#257141,#257142,#257143,#257144,#257145,#257146,#257147,
#257148,#257149,#257150,#257151,#257152),.UNSPECIFIED.,.F.,.F.,(4,3,3,3,
3,3,3,3,3,3,3,3,3,3,3,3,3,3,3,3,3,3,3,3,3,3,3,3,3,3,3,3,3,4),(1.42043608206403E-9,
8.96508236035631E-5,0.000177139225573717,0.000196453687302176,0.000222064227861251,
0.000285479098216081,0.0003490056424501,0.000361856879033412,0.000392907374604345,
0.000507356384677133,0.00059577553344614,0.000684346942743958,0.000773468971644799,
0.00078581474920867,0.000832772345389567,0.000952902380959916,0.00107741065982593,
0.001178722123813,0.00121565072790588,0.00131178235000143,0.00141569811400841,
0.00142936137630791,0.0015593159657081,0.00157162949841732,0.00165375706712266,
0.00184401976967872,0.00204137976426714,0.00212850003740968,0.00230460243517562,
0.00235744424762599,0.00259423468398172,0.002630138201466,0.00296211475105057,
0.00314325899683465),.UNSPECIFIED.);
#5317=B_SPLINE_CURVE_WITH_KNOTS('',3,(#257154,#257155,#257156,#257157,#257158,
#257159,#257160,#257161,#257162,#257163,#257164,#257165,#257166,#257167,
#257168,#257169,#257170,#257171,#257172,#257173,#257174,#257175,#257176,
#257177,#257178,#257179,#257180,#257181,#257182,#257183,#257184,#257185,
#257186,#257187,#257188,#257189,#257190,#257191,#257192,#257193,#257194,
#257195,#257196,#257197,#257198,#257199,#257200,#257201,#257202,#257203,
#257204,#257205,#257206,#257207,#257208,#257209,#257210,#257211,#257212,
#257213,#257214,#257215,#257216,#257217,#257218,#257219,#257220,#257221,
#257222,#257223,#257224,#257225,#257226,#257227,#257228,#257229,#257230,
#257231,#257232,#257233,#257234,#257235,#257236,#257237,#257238,#257239,
#257240,#257241,#257242,#257243,#257244),.UNSPECIFIED.,.F.,.F.,(4,3,3,3,
3,3,3,3,3,3,3,3,3,3,3,3,3,3,3,3,3,3,3,3,3,3,3,3,3,3,4),(7.76567327304113E-17,
0.00028555321634447,0.000553574635556241,0.000790156389930066,0.000990625082294371,
0.00101175876514238,0.00118107858470282,0.00133650434438385,0.00148689176226834,
0.00158031277986005,0.00171723652027668,0.00184679122665669,0.00192446598409234,
0.00197539097482506,0.00208289236625799,0.00218748593006637,0.0022881074172723,
0.0023115638194695,0.00237046916979006,0.00246035369911973,0.00255120401579351,
0.00263700098462238,0.00276554736475506,0.00278116187942606,0.00285032890543618,
0.0029194959314463,0.00296308646223756,0.00302598539539431,0.0030896083045167,
0.00315476369574107,0.00316062555972006),.UNSPECIFIED.);
#5318=B_SPLINE_CURVE_WITH_KNOTS('',3,(#257246,#257247,#257248,#257249,#257250,
#257251,#257252,#257253,#257254,#257255,#257256,#257257,#257258,#257259,
#257260,#257261,#257262,#257263,#257264,#257265,#257266,#257267,#257268,
#257269,#257270,#257271,#257272,#257273,#257274,#257275,#257276,#257277,
#257278,#257279,#257280,#257281,#257282,#257283,#257284,#257285,#257286,
#257287,#257288,#257289,#257290,#257291,#257292,#257293,#257294,#257295,
#257296,#257297,#257298,#257299,#257300,#257301,#257302,#257303,#257304,
#257305,#257306,#257307,#257308,#257309,#257310,#257311,#257312,#257313,
#257314,#257315,#257316,#257317,#257318,#257319,#257320,#257321,#257322,
#257323,#257324,#257325,#257326,#257327,#257328,#257329,#257330,#257331,
#257332,#257333,#257334,#257335,#257336,#257337,#257338,#257339,#257340,
#257341,#257342,#257343,#257344,#257345),.UNSPECIFIED.,.F.,.F.,(4,3,3,3,
3,3,3,3,3,3,3,3,3,3,3,3,3,3,3,3,3,3,3,3,3,3,3,3,3,3,3,3,3,4),(1.42043589704641E-9,
8.96508235406491E-5,0.000177139225437119,0.000196453687302197,0.000222064227860353,
0.000285479098225494,0.00034900564245659,0.000361856879032499,0.000392907374604361,
0.000507356384676228,0.000595775533459017,0.000684346942768234,0.000773468971677273,
0.000785814749208695,0.000832772345388566,0.000952902380893963,0.00107741065969749,
0.00117872212381303,0.00121565072790504,0.00131178235002272,0.00141569811405072,
0.00142936137630815,0.00155931596573497,0.00157162949841736,0.00165375706712212,
0.00184401976963584,0.00204137976419306,0.0021285000374072,0.00230460243515318,
0.00235744424762603,0.00259423468397992,0.00263013820146432,0.00296211475118288,
0.0031432589968347),.UNSPECIFIED.);
#5319=B_SPLINE_CURVE_WITH_KNOTS('',3,(#257347,#257348,#257349,#257350,#257351,
#257352,#257353,#257354,#257355,#257356,#257357,#257358,#257359,#257360,
#257361,#257362,#257363,#257364,#257365,#257366,#257367,#257368,#257369,
#257370,#257371,#257372,#257373,#257374,#257375,#257376,#257377,#257378,
#257379,#257380,#257381,#257382,#257383,#257384,#257385,#257386,#257387,
#257388,#257389,#257390,#257391,#257392,#257393,#257394,#257395,#257396,
#257397,#257398,#257399,#257400,#257401,#257402,#257403,#257404,#257405,
#257406,#257407,#257408,#257409,#257410,#257411,#257412,#257413,#257414,
#257415,#257416,#257417,#257418,#257419,#257420,#257421,#257422,#257423,
#257424,#257425,#257426,#257427,#257428,#257429,#257430,#257431,#257432,
#257433,#257434,#257435,#257436,#257437,#257438,#257439,#257440,#257441,
#257442,#257443,#257444,#257445,#257446),.UNSPECIFIED.,.F.,.F.,(4,3,3,3,
3,3,3,3,3,3,3,3,3,3,3,3,3,3,3,3,3,3,3,3,3,3,3,3,3,3,3,3,3,4),(3.46944695195361E-18,
0.000232066433521906,0.000444177579881847,0.000518385099121857,0.00073410278654322,
0.000790156389930058,0.00099348773274801,0.00102299023054891,0.00119225943856017,
0.0013476470003594,0.00150263588856866,0.00158031277986011,0.00171536369188439,
0.00184243086343882,0.00194346242503234,0.00197539097482514,0.00208159421173027,
0.0021848752532145,0.00228393672704159,0.0023319957435323,0.00237046916979017,
0.00246124899502891,0.00255227503603492,0.00264431970440927,0.00265740253517351,
0.0027655473647552,0.00280202928404987,0.00287180839700916,0.00294158750996845,
0.00296308646223771,0.00302593425587023,0.00308943159920767,0.00315434926415385,
0.00316062418320325),.UNSPECIFIED.);
#5320=B_SPLINE_CURVE_WITH_KNOTS('',3,(#257448,#257449,#257450,#257451,#257452,
#257453,#257454,#257455,#257456,#257457,#257458,#257459,#257460,#257461,
#257462,#257463,#257464,#257465,#257466,#257467,#257468,#257469,#257470,
#257471,#257472,#257473,#257474,#257475,#257476,#257477,#257478,#257479,
#257480,#257481,#257482,#257483,#257484,#257485,#257486,#257487,#257488,
#257489,#257490,#257491,#257492,#257493,#257494,#257495,#257496,#257497,
#257498,#257499,#257500,#257501,#257502,#257503,#257504,#257505,#257506,
#257507,#257508,#257509,#257510,#257511,#257512,#257513,#257514,#257515,
#257516,#257517,#257518,#257519,#257520,#257521,#257522,#257523,#257524,
#257525,#257526,#257527,#257528,#257529,#257530,#257531,#257532,#257533,
#257534,#257535,#257536,#257537,#257538,#257539,#257540,#257541,#257542,
#257543,#257544,#257545,#257546,#257547),.UNSPECIFIED.,.F.,.F.,(4,3,3,3,
3,3,3,3,3,3,3,3,3,3,3,3,3,3,3,3,3,3,3,3,3,3,3,3,3,3,3,3,3,4),(1.42043598509044E-9,
8.96508235342264E-5,0.00017713922542495,0.000196453687302173,0.000222064227861238,
0.000285479098223288,0.000349005642442205,0.00036185687903336,0.000392907374604334,
0.000507356384677039,0.000595775533454771,0.000684346942758704,0.000773468971665902,
0.000785814749208657,0.000832772345389472,0.00095290238088768,0.0010774106596845,
0.00117872212381298,0.00121565072790591,0.00131178235000832,0.00141569811402118,
0.0014293613763088,0.0015593159657519,0.0015716294984173,0.00165375706712255,
0.00184401976964395,0.0020413797642039,0.00212850003740835,0.00230460243515425,
0.00235744424762595,0.00259423468409489,0.00263013820146402,0.00296211475216053,
0.0031432589968346),.UNSPECIFIED.);
#5321=B_SPLINE_CURVE_WITH_KNOTS('',3,(#257552,#257553,#257554,#257555,#257556,
#257557,#257558,#257559,#257560,#257561,#257562,#257563,#257564,#257565,
#257566,#257567,#257568,#257569,#257570,#257571,#257572,#257573,#257574,
#257575,#257576,#257577,#257578,#257579,#257580,#257581,#257582,#257583,
#257584,#257585,#257586,#257587,#257588,#257589,#257590,#257591,#257592,
#257593,#257594,#257595,#257596,#257597,#257598,#257599,#257600,#257601,
#257602,#257603,#257604,#257605,#257606,#257607,#257608,#257609,#257610,
#257611,#257612,#257613,#257614,#257615,#257616,#257617,#257618,#257619,
#257620,#257621,#257622,#257623,#257624,#257625,#257626,#257627,#257628,
#257629,#257630,#257631,#257632,#257633,#257634,#257635,#257636,#257637,
#257638,#257639,#257640,#257641,#257642,#257643,#257644,#257645,#257646,
#257647,#257648,#257649,#257650,#257651),.UNSPECIFIED.,.F.,.F.,(4,3,3,3,
3,3,3,3,3,3,3,3,3,3,3,3,3,3,3,3,3,3,3,3,3,3,3,3,3,3,3,3,3,4),(6.93889390390723E-18,
0.000232066433641197,0.000444177580043925,0.000518385099123124,0.00073410278665711,
0.000790156389930058,0.000993487732784391,0.00102299023054913,0.00119225943858464,
0.00134764700041078,0.00150263588856873,0.00158031277986011,0.0017153636919325,
0.00184243086354218,0.00194346242503232,0.00197539097482513,0.00208159421175262,
0.00218487525326351,0.00228393672712271,0.00233199574353222,0.00237046916979016,
0.00246124899502871,0.00255227503603373,0.00264431970440758,0.0026574025351733,
0.00276554736475518,0.0028020292840497,0.00287180839700904,0.00294158750996837,
0.0029630864622377,0.00302593425586324,0.00308943159919611,0.00315434926414153,
0.00316062418320342),.UNSPECIFIED.);
#5322=B_SPLINE_CURVE_WITH_KNOTS('',3,(#257719,#257720,#257721,#257722,#257723,
#257724,#257725,#257726,#257727,#257728,#257729,#257730,#257731,#257732,
#257733,#257734,#257735,#257736,#257737,#257738,#257739,#257740,#257741,
#257742,#257743,#257744,#257745,#257746,#257747,#257748,#257749,#257750,
#257751,#257752,#257753,#257754,#257755,#257756,#257757,#257758,#257759,
#257760,#257761,#257762,#257763,#257764,#257765,#257766,#257767,#257768,
#257769,#257770,#257771,#257772,#257773,#257774,#257775,#257776,#257777,
#257778,#257779,#257780,#257781,#257782,#257783,#257784,#257785,#257786,
#257787,#257788,#257789,#257790,#257791,#257792,#257793,#257794,#257795,
#257796,#257797,#257798,#257799,#257800,#257801,#257802,#257803,#257804,
#257805,#257806,#257807,#257808,#257809,#257810,#257811,#257812,#257813,
#257814,#257815,#257816,#257817,#257818,#257819,#257820,#257821,#257822,
#257823,#257824,#257825,#257826,#257827,#257828,#257829,#257830,#257831,
#257832,#257833,#257834,#257835,#257836,#257837,#257838,#257839,#257840,
#257841,#257842,#257843,#257844,#257845,#257846,#257847,#257848,#257849,
#257850,#257851,#257852,#257853,#257854,#257855,#257856,#257857,#257858,
#257859,#257860,#257861,#257862,#257863,#257864,#257865,#257866,#257867,
#257868,#257869,#257870,#257871,#257872,#257873,#257874,#257875),
 .UNSPECIFIED.,.F.,.F.,(4,3,3,3,3,3,3,3,3,3,3,3,3,3,3,3,3,3,3,3,3,3,3,3,
3,3,3,3,3,3,3,3,3,3,3,3,3,3,3,3,3,3,3,3,3,3,3,3,3,3,3,3,4),(6.7720902829718E-17,
4.10182404401297E-5,4.87365934461908E-5,8.48991743434339E-5,0.000100950649804241,
0.000144177502975245,0.00015950443871374,0.000183552069859812,0.000204873519796485,
0.000207599701005883,0.000228271330673476,0.000247545550387866,0.000265562240286856,
0.00028198101272654,0.00028897409501864,0.000314246599144076,0.000319008877427412,
0.000335084346478968,0.000341191974140351,0.000360114345590793,0.000376222888385349,
0.000387536967904427,0.000398062148035578,0.000398761096784253,0.00040134372044755,
0.000415942457382944,0.000428117175977391,0.000438082433319717,0.000455134767349359,
0.000469444387012387,0.000478513316141094,0.000488773476917098,0.000516028797194734,
0.000543665383177674,0.000571301969160615,0.000614049546779864,0.00063801775485477,
0.000716147133287823,0.000844915617942006,0.000857475220032229,0.000957026632282125,
0.00114329303177871,0.00127603550970948,0.0014210220315045,0.00160971753355524,
0.00179821625845706,0.0019140532645642,0.00198770968410965,0.00213898443966606,
0.0022789813273605,0.00241552617338971,0.00253842863988512,0.00255207101941893),
 .UNSPECIFIED.);
#5323=B_SPLINE_CURVE_WITH_KNOTS('',3,(#257876,#257877,#257878,#257879,#257880,
#257881,#257882,#257883,#257884,#257885,#257886,#257887,#257888),
 .UNSPECIFIED.,.F.,.F.,(4,3,3,3,4),(2.95802686519878E-17,6.33504396955935E-5,
0.000127359484775983,0.000192332933960853,0.000199794734077019),
 .UNSPECIFIED.);
#5324=B_SPLINE_CURVE_WITH_KNOTS('',3,(#257953,#257954,#257955,#257956,#257957,
#257958,#257959,#257960,#257961,#257962,#257963,#257964,#257965),
 .UNSPECIFIED.,.F.,.F.,(4,3,3,3,4),(1.30709403380831E-8,6.47809505539985E-5,
0.000128843980536247,0.000191999731800387,0.000199807394155651),
 .UNSPECIFIED.);
#5325=B_SPLINE_CURVE_WITH_KNOTS('',3,(#257966,#257967,#257968,#257969,#257970,
#257971,#257972,#257973,#257974,#257975,#257976,#257977,#257978,#257979,
#257980,#257981,#257982,#257983,#257984,#257985,#257986,#257987,#257988,
#257989,#257990,#257991,#257992,#257993,#257994,#257995,#257996,#257997,
#257998,#257999,#258000,#258001,#258002,#258003,#258004,#258005,#258006,
#258007,#258008,#258009,#258010,#258011,#258012,#258013,#258014,#258015,
#258016,#258017,#258018,#258019,#258020,#258021,#258022,#258023,#258024,
#258025,#258026,#258027,#258028,#258029,#258030,#258031,#258032,#258033,
#258034,#258035,#258036,#258037,#258038,#258039,#258040,#258041,#258042,
#258043,#258044,#258045,#258046,#258047,#258048,#258049,#258050,#258051,
#258052,#258053,#258054,#258055,#258056,#258057,#258058,#258059,#258060,
#258061,#258062,#258063,#258064,#258065,#258066,#258067,#258068,#258069,
#258070,#258071,#258072,#258073,#258074,#258075,#258076,#258077,#258078,
#258079,#258080,#258081,#258082,#258083,#258084,#258085,#258086,#258087,
#258088,#258089,#258090,#258091,#258092,#258093,#258094,#258095,#258096,
#258097,#258098,#258099,#258100,#258101,#258102,#258103,#258104,#258105,
#258106,#258107,#258108,#258109,#258110,#258111,#258112,#258113,#258114,
#258115,#258116,#258117,#258118,#258119),.UNSPECIFIED.,.F.,.F.,(4,3,3,3,
3,3,3,3,3,3,3,3,3,3,3,3,3,3,3,3,3,3,3,3,3,3,3,3,3,3,3,3,3,3,3,3,3,3,3,3,
3,3,3,3,3,3,3,3,3,3,3,4),(0.,0.000185828670303492,0.000382716193704216,
0.000559934895967205,0.000631076048494892,0.000828487317476088,0.00103761547331349,
0.00111698223038901,0.00126215209698978,0.00146547701524327,0.00157769012123723,
0.00167319966665239,0.00179700293119311,0.00181236538820063,0.00189322814548469,
0.0019236575551527,0.00195311374872379,0.0019744410311806,0.00199411982899787,
0.00201373802954043,0.00203411668352692,0.00203842287855105,0.00205099715760843,
0.00207138344075605,0.00209424343179354,0.0021061580023323,0.00212252899831673,
0.00214057390931081,0.00215045406625544,0.00216323449344539,0.00217718293490172,
0.00219274290031516,0.00220789813799093,0.00220876616973217,0.00222335836349227,
0.00224350969408024,0.0022482563035986,0.00226071864757904,0.00227459317807681,
0.00228941445633327,0.00230590048913228,0.00231448813766505,0.00233284153072107,
0.0023534591125159,0.00236653518185591,0.00241507181483341,0.00241846009663411,
0.0024531315509032,0.00247060413398639,0.0025112586054267,0.00252226520021835,
0.00252430419397965),.UNSPECIFIED.);
#5326=B_SPLINE_CURVE_WITH_KNOTS('',3,(#258187,#258188,#258189,#258190,#258191,
#258192,#258193,#258194,#258195,#258196,#258197,#258198,#258199,#258200,
#258201,#258202,#258203,#258204,#258205,#258206,#258207,#258208,#258209,
#258210,#258211,#258212,#258213,#258214,#258215,#258216,#258217,#258218,
#258219,#258220,#258221,#258222,#258223,#258224,#258225,#258226,#258227,
#258228,#258229,#258230,#258231,#258232,#258233,#258234,#258235,#258236,
#258237,#258238,#258239,#258240,#258241,#258242,#258243,#258244,#258245,
#258246,#258247,#258248,#258249,#258250,#258251,#258252,#258253,#258254,
#258255,#258256,#258257,#258258,#258259,#258260,#258261,#258262,#258263,
#258264,#258265,#258266,#258267,#258268,#258269,#258270,#258271,#258272,
#258273,#258274,#258275,#258276,#258277,#258278,#258279,#258280,#258281,
#258282,#258283,#258284,#258285,#258286,#258287,#258288,#258289,#258290,
#258291,#258292,#258293,#258294,#258295,#258296,#258297,#258298,#258299,
#258300,#258301,#258302,#258303,#258304,#258305,#258306,#258307,#258308,
#258309,#258310,#258311,#258312,#258313,#258314,#258315,#258316,#258317,
#258318,#258319,#258320,#258321,#258322,#258323,#258324,#258325,#258326,
#258327,#258328,#258329,#258330,#258331,#258332,#258333,#258334,#258335,
#258336,#258337,#258338,#258339,#258340,#258341,#258342,#258343),
 .UNSPECIFIED.,.F.,.F.,(4,3,3,3,3,3,3,3,3,3,3,3,3,3,3,3,3,3,3,3,3,3,3,3,
3,3,3,3,3,3,3,3,3,3,3,3,3,3,3,3,3,3,3,3,3,3,3,3,3,3,3,3,4),(2.4532694666934E-16,
4.10182404382943E-5,4.87365934320212E-5,8.48991743424062E-5,0.000100950649789678,
0.000144177502945797,0.000159504438714265,0.000183552069852738,0.000204873519784471,
0.00020759970099121,0.000228271330655785,0.000247545550365401,0.000265562240258363,
0.00028198101269087,0.00028897409500906,0.000314246599079761,0.000319008877428285,
0.000335084346452271,0.000341191974135023,0.000360114345606934,0.000376222888380103,
0.00038753696789393,0.000398062148021026,0.00039876109678529,0.000401343720445582,
0.000415942457351562,0.000428117175926856,0.000438082433318889,0.00045513476735202,
0.000469444387017119,0.000478513316142295,0.000488773476917066,0.000516028797212078,
0.000543665383186523,0.000571301969160969,0.000614049546817563,0.000638017754856327,
0.000716147133288671,0.000844915617965103,0.000857475220033525,0.000957026632284375,
0.00114329303187666,0.00127603550971242,0.00142102203150686,0.00160971753352521,
0.0017982162583827,0.0019140532645685,0.00198770968411401,0.00213898444013934,
0.00227898132821245,0.00241552617381852,0.00253842864049211,0.00255207101942458),
 .UNSPECIFIED.);
#5327=B_SPLINE_CURVE_WITH_KNOTS('',3,(#258344,#258345,#258346,#258347,#258348,
#258349,#258350,#258351,#258352,#258353,#258354,#258355,#258356),
 .UNSPECIFIED.,.F.,.F.,(4,3,3,3,4),(4.9065389333868E-18,6.3350439619856E-5,
0.000127359484550393,0.000192332933484367,0.000199794734076953),
 .UNSPECIFIED.);
#5328=B_SPLINE_CURVE_WITH_KNOTS('',3,(#258421,#258422,#258423,#258424,#258425,
#258426,#258427,#258428,#258429,#258430,#258431,#258432,#258433),
 .UNSPECIFIED.,.F.,.F.,(4,3,3,3,4),(1.30709403943339E-8,6.47809508571854E-5,
0.000128843981032926,0.000191999732342699,0.00019980739415557),
 .UNSPECIFIED.);
#5329=B_SPLINE_CURVE_WITH_KNOTS('',3,(#258434,#258435,#258436,#258437,#258438,
#258439,#258440,#258441,#258442,#258443,#258444,#258445,#258446,#258447,
#258448,#258449,#258450,#258451,#258452,#258453,#258454,#258455,#258456,
#258457,#258458,#258459,#258460,#258461,#258462,#258463,#258464,#258465,
#258466,#258467,#258468,#258469,#258470,#258471,#258472,#258473,#258474,
#258475,#258476,#258477,#258478,#258479,#258480,#258481,#258482,#258483,
#258484,#258485,#258486,#258487,#258488,#258489,#258490,#258491,#258492,
#258493,#258494,#258495,#258496,#258497,#258498,#258499,#258500,#258501,
#258502,#258503,#258504,#258505,#258506,#258507,#258508,#258509,#258510,
#258511,#258512,#258513,#258514,#258515,#258516,#258517,#258518,#258519,
#258520,#258521,#258522,#258523,#258524,#258525,#258526,#258527,#258528,
#258529,#258530,#258531,#258532,#258533,#258534,#258535,#258536,#258537,
#258538,#258539,#258540,#258541,#258542,#258543,#258544,#258545,#258546,
#258547,#258548,#258549,#258550,#258551,#258552,#258553,#258554,#258555,
#258556,#258557,#258558,#258559,#258560,#258561,#258562,#258563,#258564,
#258565,#258566,#258567,#258568,#258569,#258570,#258571,#258572,#258573,
#258574,#258575,#258576,#258577,#258578,#258579,#258580,#258581,#258582,
#258583,#258584,#258585,#258586,#258587),.UNSPECIFIED.,.F.,.F.,(4,3,3,3,
3,3,3,3,3,3,3,3,3,3,3,3,3,3,3,3,3,3,3,3,3,3,3,3,3,3,3,3,3,3,3,3,3,3,3,3,
3,3,3,3,3,3,3,3,3,3,3,4),(0.,0.000185828671060948,0.00038271619533701,0.000559934896067518,
0.000631076048494951,0.000828487317448596,0.00103761547327565,0.00111698223059055,
0.0012621520969899,0.00146547701548244,0.00157769012123739,0.00167319966695433,
0.00179700293135962,0.00181236538852903,0.00189322814548488,0.00192365755511324,
0.00195311374909541,0.00197444103160466,0.00199411982937103,0.00201373802987178,
0.00203411668383433,0.00203842287913242,0.00205099715760863,0.00207138344065033,
0.00209424343157988,0.00210615800318399,0.00212252899910065,0.00214057391002469,
0.00215045406732086,0.00216323449445623,0.00217718293585703,0.00219274290122226,
0.00220789813945474,0.00220876616973239,0.00222335836372349,0.00224350969435737,
0.00224825630573298,0.00226071864973988,0.00227459318032408,0.00228941445870785,
0.00230590049174731,0.00231448814155603,0.00233284153412959,0.00235345911575492,
0.00236653518185614,0.00241507181112009,0.00241846010128728,0.00245313155701541,
0.00247060413857423,0.00251125861000287,0.00252226520475691,0.0025243041939799),
 .UNSPECIFIED.);
#5330=B_SPLINE_CURVE_WITH_KNOTS('',3,(#258655,#258656,#258657,#258658,#258659,
#258660,#258661,#258662,#258663,#258664,#258665,#258666,#258667,#258668,
#258669,#258670,#258671,#258672,#258673,#258674,#258675,#258676,#258677,
#258678,#258679,#258680,#258681,#258682,#258683,#258684,#258685,#258686,
#258687,#258688,#258689,#258690,#258691,#258692,#258693,#258694,#258695,
#258696,#258697,#258698,#258699,#258700,#258701,#258702,#258703,#258704,
#258705,#258706,#258707,#258708,#258709,#258710,#258711,#258712,#258713,
#258714,#258715,#258716,#258717,#258718,#258719,#258720,#258721,#258722,
#258723,#258724,#258725,#258726,#258727,#258728,#258729,#258730,#258731,
#258732,#258733,#258734,#258735,#258736,#258737,#258738,#258739,#258740,
#258741,#258742,#258743,#258744,#258745,#258746,#258747,#258748,#258749,
#258750,#258751,#258752,#258753,#258754,#258755,#258756,#258757,#258758,
#258759,#258760,#258761,#258762,#258763,#258764,#258765,#258766,#258767,
#258768,#258769,#258770,#258771,#258772,#258773,#258774,#258775,#258776,
#258777,#258778,#258779,#258780,#258781,#258782,#258783,#258784,#258785,
#258786,#258787,#258788,#258789,#258790,#258791,#258792,#258793,#258794,
#258795,#258796,#258797,#258798,#258799,#258800,#258801,#258802,#258803,
#258804,#258805,#258806,#258807,#258808,#258809,#258810,#258811),
 .UNSPECIFIED.,.F.,.F.,(4,3,3,3,3,3,3,3,3,3,3,3,3,3,3,3,3,3,3,3,3,3,3,3,
3,3,3,3,3,3,3,3,3,3,3,3,3,3,3,3,3,3,3,3,3,3,3,3,3,3,3,3,4),(4.18021567944388E-16,
4.10182404324863E-5,4.8736593467773E-5,8.48991743663496E-5,0.000100950649826721,
0.000144177502986782,0.000159504438714103,0.000183552069870851,0.000204873519798632,
0.000207599701027599,0.000228271330692523,0.000247545550402923,0.000265562240297104,
0.000281981012731784,0.00028897409503117,0.000314246599158208,0.000319008877427789,
0.000335084346479877,0.000341191974148699,0.000360114345617055,0.00037622288839528,
0.000387536967911221,0.000398062148039941,0.000398761096784631,0.000401343720451845,
0.000415942457358753,0.000428117175935046,0.000438082433322659,0.000455134767347245,
0.000469444387007091,0.000478513316141474,0.00048877347691912,0.000516028797196325,
0.000543665383179294,0.000571301969162262,0.000614049546796093,0.000638017754855134,
0.00071614713328926,0.00084491561809254,0.000857475220033438,0.000957026632282486,
0.00114329303185101,0.00127603550970984,0.00142102203150565,0.00160971753353858,
0.00179821625839819,0.00191405326456454,0.00198770968411041,0.00213898443977125,
0.00227898132754153,0.00241552617348039,0.00253842863999955,0.00255207101941925),
 .UNSPECIFIED.);
#5331=B_SPLINE_CURVE_WITH_KNOTS('',3,(#258812,#258813,#258814,#258815,#258816,
#258817,#258818,#258819,#258820,#258821,#258822,#258823,#258824),
 .UNSPECIFIED.,.F.,.F.,(4,3,3,3,4),(0.,6.33504396296269E-5,0.000127359484566964,
0.00019233293350393,0.000199794734076948),.UNSPECIFIED.);
#5332=B_SPLINE_CURVE_WITH_KNOTS('',3,(#258883,#258884,#258885,#258886,#258887,
#258888,#258889,#258890,#258891,#258892,#258893,#258894,#258895),
 .UNSPECIFIED.,.F.,.F.,(4,3,3,3,4),(2.22293795268E-9,6.4770213458298E-5,
0.00012883335096098,0.00019198917072549,0.000199807394155362),
 .UNSPECIFIED.);
#5333=B_SPLINE_CURVE_WITH_KNOTS('',3,(#258897,#258898,#258899,#258900,#258901,
#258902,#258903,#258904,#258905,#258906,#258907,#258908,#258909,#258910,
#258911,#258912,#258913,#258914,#258915,#258916,#258917,#258918,#258919,
#258920,#258921,#258922,#258923,#258924,#258925,#258926,#258927,#258928,
#258929,#258930,#258931,#258932,#258933,#258934,#258935,#258936,#258937,
#258938,#258939,#258940,#258941,#258942,#258943,#258944,#258945,#258946,
#258947,#258948,#258949,#258950,#258951,#258952,#258953,#258954,#258955,
#258956,#258957,#258958,#258959,#258960,#258961,#258962,#258963,#258964,
#258965,#258966,#258967,#258968,#258969,#258970,#258971,#258972,#258973,
#258974,#258975,#258976,#258977,#258978,#258979,#258980,#258981,#258982,
#258983,#258984,#258985,#258986,#258987,#258988,#258989,#258990,#258991,
#258992,#258993,#258994,#258995,#258996,#258997,#258998,#258999,#259000,
#259001,#259002,#259003,#259004,#259005),.UNSPECIFIED.,.F.,.F.,(4,3,3,3,
3,3,3,3,3,3,3,3,3,3,3,3,3,3,3,3,3,3,3,3,3,3,3,3,3,3,3,3,3,3,3,3,4),(0.,
0.000141625141903644,0.00028605408553883,0.000431017935692696,0.000576069710995619,
0.000624076123138545,0.00079602838556846,0.00096948848303351,0.00114602454208786,
0.00124815224627709,0.0013835380435854,0.00152204450729419,0.00156019030784637,
0.00164202290670349,0.00172485230055762,0.00180786034566625,0.00187222836941565,
0.00191560917303388,0.00195712980570751,0.00199416155797507,0.00202824740020027,
0.00206354484838072,0.00206596024805153,0.00210374901736408,0.00210625691559258,
0.00214321751039884,0.00218002903358911,0.00218426643098488,0.00222069855051545,
0.00226227594637718,0.00227202713580122,0.00228055942654725,0.00233446236996583,
0.00234028546176949,0.00240654563051095,0.00247393114839013,0.0024963044925541),
 .UNSPECIFIED.);
#5334=B_SPLINE_CURVE_WITH_KNOTS('',3,(#259068,#259069,#259070,#259071,#259072,
#259073,#259074,#259075,#259076,#259077,#259078,#259079,#259080),
 .UNSPECIFIED.,.F.,.F.,(4,3,3,3,4),(1.30709404307573E-8,6.47809509226653E-5,
0.000128843981149524,0.000191999732492249,0.000199807394155828),
 .UNSPECIFIED.);
#5335=B_SPLINE_CURVE_WITH_KNOTS('',3,(#259081,#259082,#259083,#259084,#259085,
#259086,#259087,#259088,#259089,#259090,#259091,#259092,#259093,#259094,
#259095,#259096,#259097,#259098,#259099,#259100,#259101,#259102,#259103,
#259104,#259105,#259106,#259107,#259108,#259109,#259110,#259111,#259112,
#259113,#259114,#259115,#259116,#259117,#259118,#259119,#259120,#259121,
#259122,#259123,#259124,#259125,#259126,#259127,#259128,#259129,#259130,
#259131,#259132,#259133,#259134,#259135,#259136,#259137,#259138,#259139,
#259140,#259141,#259142,#259143,#259144,#259145,#259146,#259147,#259148,
#259149,#259150,#259151,#259152,#259153,#259154,#259155,#259156,#259157,
#259158,#259159,#259160,#259161,#259162,#259163,#259164,#259165,#259166,
#259167,#259168,#259169,#259170,#259171,#259172,#259173,#259174,#259175,
#259176,#259177,#259178,#259179,#259180,#259181,#259182,#259183,#259184,
#259185,#259186,#259187,#259188,#259189,#259190,#259191,#259192,#259193,
#259194,#259195,#259196,#259197,#259198,#259199,#259200,#259201,#259202,
#259203,#259204,#259205,#259206,#259207,#259208,#259209,#259210,#259211,
#259212,#259213,#259214,#259215,#259216,#259217,#259218,#259219,#259220,
#259221,#259222,#259223,#259224,#259225,#259226,#259227,#259228,#259229,
#259230,#259231,#259232,#259233,#259234),.UNSPECIFIED.,.F.,.F.,(4,3,3,3,
3,3,3,3,3,3,3,3,3,3,3,3,3,3,3,3,3,3,3,3,3,3,3,3,3,3,3,3,3,3,3,3,3,3,3,3,
3,3,3,3,3,3,3,3,3,3,3,4),(0.,0.000185828671079349,0.000382716195553923,
0.000559934894934763,0.000631076048495516,0.000828487317318044,0.00103761547308088,
0.00111698222831438,0.00126215209699103,0.00146547701368322,0.00157769012123879,
0.00167319966354923,0.00179700292900438,0.00181236538482168,0.00189322814548654,
0.00192365755549693,0.00195311374490067,0.00197444102681827,0.0019941198250935,
0.0020137380259943,0.0020341166801399,0.00203842287257104,0.00205099715761042,
0.00207138344176387,0.00209424343380434,0.00210615799356767,0.0021225289902399,
0.00214057390194255,0.00215045405528944,0.00216323448310569,0.00217718292521093,
0.00219274289121646,0.00220789812292523,0.0022087661697343,0.00222335836113128,
0.0022435096912273,0.00224825628163283,0.0022607186253873,0.00227459315504108,
0.00228941443202955,0.00230590046238967,0.002314488097619,0.00233284149563267,
0.00235345907916819,0.00236653518185818,0.00241507185297962,0.0024184600487372,
0.00245313148794348,0.00247060408675825,0.00251125855826495,0.00252226515349361,
0.00252430419398206),.UNSPECIFIED.);
#5336=B_SPLINE_CURVE_WITH_KNOTS('',3,(#259305,#259306,#259307,#259308,#259309,
#259310,#259311,#259312,#259313,#259314,#259315,#259316,#259317,#259318,
#259319,#259320,#259321,#259322,#259323,#259324,#259325,#259326,#259327,
#259328,#259329,#259330,#259331,#259332,#259333,#259334,#259335,#259336,
#259337,#259338,#259339,#259340,#259341,#259342,#259343,#259344,#259345,
#259346,#259347,#259348,#259349,#259350,#259351,#259352,#259353,#259354,
#259355,#259356,#259357,#259358,#259359,#259360,#259361,#259362,#259363,
#259364,#259365,#259366,#259367,#259368,#259369,#259370,#259371,#259372,
#259373,#259374,#259375,#259376,#259377,#259378,#259379,#259380,#259381,
#259382,#259383,#259384,#259385,#259386,#259387,#259388,#259389,#259390,
#259391,#259392,#259393,#259394,#259395,#259396,#259397,#259398,#259399,
#259400,#259401,#259402,#259403,#259404,#259405,#259406,#259407,#259408,
#259409,#259410,#259411,#259412,#259413,#259414,#259415,#259416,#259417,
#259418,#259419,#259420,#259421,#259422,#259423,#259424,#259425,#259426,
#259427,#259428,#259429,#259430,#259431,#259432,#259433,#259434,#259435,
#259436,#259437,#259438,#259439,#259440,#259441,#259442,#259443,#259444,
#259445,#259446,#259447,#259448,#259449,#259450,#259451,#259452,#259453,
#259454,#259455,#259456,#259457,#259458,#259459,#259460,#259461),
 .UNSPECIFIED.,.F.,.F.,(4,3,3,3,3,3,3,3,3,3,3,3,3,3,3,3,3,3,3,3,3,3,3,3,
3,3,3,3,3,3,3,3,3,3,3,3,3,3,3,3,3,3,3,3,3,3,3,3,3,3,3,3,4),(1.59179194089066E-16,
4.10182404321299E-5,4.87365934503859E-5,8.48991743553393E-5,0.000100950649807767,
0.000144177502998116,0.00015950443871382,0.000183552069860929,0.000204873519804175,
0.000207599701008038,0.000228271330675712,0.000247545550391478,0.000265562240292495,
0.000281981012734991,0.000288974095020833,0.000314246599120257,0.000319008877427481,
0.000335084346465828,0.000341191974142289,0.0003601143455919,0.000376222888387497,
0.000387536967906843,0.000398062148038267,0.000398761096784301,0.000401343720448768,
0.000415942457365449,0.000428117175948292,0.000438082433320561,0.000455134767335398,
0.000469444386988523,0.000478513316141121,0.000488773476917633,0.000516028797205843,
0.000543665383183412,0.000571301969160981,0.000614049546779688,0.000638017754854762,
0.000716147133288069,0.000844915617838834,0.000857475220032411,0.000957026632282044,
0.00114329303175841,0.00127603550970933,0.00142102203150452,0.00160971753356947,
0.00179821625849527,0.0019140532645639,0.00198770968410954,0.00213898444007436,
0.00227898132810696,0.00241552617376272,0.00253842864042649,0.00255207101941848),
 .UNSPECIFIED.);
#5337=B_SPLINE_CURVE_WITH_KNOTS('',3,(#259462,#259463,#259464,#259465,#259466,
#259467,#259468,#259469,#259470,#259471,#259472,#259473,#259474),
 .UNSPECIFIED.,.F.,.F.,(4,3,3,3,4),(0.,6.33504393148245E-5,0.000127359483688777,
0.00019233293172222,0.000199794734076686),.UNSPECIFIED.);
#5338=B_SPLINE_CURVE_WITH_KNOTS('',3,(#259487,#259488,#259489,#259490,#259491,
#259492,#259493,#259494,#259495,#259496,#259497,#259498,#259499,#259500,
#259501,#259502,#259503,#259504,#259505,#259506,#259507,#259508,#259509,
#259510,#259511,#259512,#259513,#259514,#259515,#259516,#259517,#259518,
#259519,#259520,#259521,#259522,#259523,#259524,#259525,#259526,#259527,
#259528,#259529,#259530,#259531,#259532,#259533,#259534,#259535,#259536,
#259537,#259538),.UNSPECIFIED.,.F.,.F.,(4,3,3,3,3,3,3,3,3,3,3,3,3,3,3,3,
3,4),(0.,0.000158823224858671,0.000317052051105456,0.000468924589491904,
0.00047967179401345,0.000658381832507577,0.000717650779103897,0.000878959899787774,
0.000937849178983809,0.000953578178040417,0.00118717940744276,0.00135200974701517,
0.00140677376847571,0.00141855942378738,0.00156529908011683,0.00171075963989374,
0.0018547794947342,0.00187569835796762),.UNSPECIFIED.);
#5339=B_SPLINE_CURVE_WITH_KNOTS('',3,(#259554,#259555,#259556,#259557,#259558,
#259559),.UNSPECIFIED.,.F.,.F.,(4,2,4),(-0.0664084835399893,-0.0331810811129581,
-2.20931276191819E-6),.UNSPECIFIED.);
#5340=B_SPLINE_CURVE_WITH_KNOTS('',3,(#259572,#259573,#259574,#259575,#259576,
#259577,#259578,#259579,#259580,#259581,#259582,#259583,#259584,#259585,
#259586,#259587,#259588,#259589,#259590,#259591,#259592,#259593,#259594,
#259595,#259596,#259597,#259598,#259599,#259600,#259601,#259602,#259603,
#259604,#259605,#259606,#259607,#259608,#259609,#259610,#259611),
 .UNSPECIFIED.,.F.,.F.,(4,3,3,3,3,3,3,3,3,3,3,3,3,4),(0.,0.000161852329700689,
0.000326653855066742,0.000456473147090736,0.000468231828707601,0.000687452602017532,
0.000863637906863081,0.000920751357275229,0.000936463657415201,0.00115607960829242,
0.0013377019175669,0.00139315075344184,0.00168563754506796,0.00187292731483044),
 .UNSPECIFIED.);
#5341=B_SPLINE_CURVE_WITH_KNOTS('',3,(#259627,#259628,#259629,#259630,#259631,
#259632),.UNSPECIFIED.,.F.,.F.,(4,2,4),(-0.0663140791229485,-0.0332720824825186,
-2.08023336209506E-7),.UNSPECIFIED.);
#5342=B_SPLINE_CURVE_WITH_KNOTS('',3,(#259715,#259716,#259717,#259718,#259719,
#259720,#259721,#259722,#259723,#259724),.UNSPECIFIED.,.F.,.F.,(4,3,3,4),
(-2.45811799075953E-5,0.000216663649658451,0.000460938450737844,0.000512405873606687),
 .UNSPECIFIED.);
#5343=B_SPLINE_CURVE_WITH_KNOTS('',3,(#260836,#260837,#260838,#260839,#260840,
#260841,#260842,#260843,#260844,#260845,#260846,#260847,#260848,#260849),
 .UNSPECIFIED.,.F.,.F.,(4,2,2,2,2,2,4),(0.471695282412039,0.547619803692722,
0.63289106477561,0.74233944143791,0.840749628642468,0.94339056482327,0.944354806358975),
 .UNSPECIFIED.);
#5344=B_SPLINE_CURVE_WITH_KNOTS('',3,(#260894,#260895,#260896,#260897,#260898,
#260899,#260900,#260901,#260902,#260903,#260904,#260905,#260906,#260907),
 .UNSPECIFIED.,.F.,.F.,(4,2,2,2,2,2,4),(-0.471695282403551,-0.395770761124079,
-0.31049950004257,-0.201051123381967,-0.102640936178941,0.,0.000964241535706043),
 .UNSPECIFIED.);
#5345=B_SPLINE_CURVE_WITH_KNOTS('',3,(#260997,#260998,#260999,#261000,#261001,
#261002,#261003,#261004,#261005,#261006,#261007,#261008,#261009,#261010,
#261011,#261012,#261013,#261014,#261015,#261016,#261017,#261018,#261019,
#261020,#261021,#261022,#261023,#261024,#261025,#261026,#261027,#261028,
#261029,#261030,#261031,#261032,#261033,#261034,#261035,#261036,#261037,
#261038,#261039,#261040,#261041,#261042,#261043,#261044,#261045,#261046,
#261047,#261048,#261049,#261050,#261051,#261052,#261053,#261054,#261055,
#261056,#261057,#261058,#261059,#261060,#261061,#261062,#261063,#261064,
#261065,#261066,#261067,#261068,#261069,#261070,#261071,#261072,#261073,
#261074,#261075,#261076,#261077,#261078,#261079,#261080,#261081,#261082,
#261083,#261084,#261085,#261086,#261087,#261088,#261089,#261090,#261091,
#261092,#261093,#261094,#261095,#261096,#261097,#261098,#261099,#261100,
#261101,#261102,#261103,#261104,#261105,#261106,#261107,#261108,#261109,
#261110,#261111,#261112,#261113,#261114,#261115,#261116,#261117,#261118,
#261119,#261120,#261121,#261122,#261123,#261124,#261125,#261126,#261127,
#261128,#261129,#261130,#261131,#261132,#261133,#261134,#261135,#261136,
#261137,#261138,#261139,#261140,#261141,#261142,#261143,#261144,#261145,
#261146,#261147,#261148,#261149,#261150,#261151,#261152,#261153,#261154,
#261155,#261156,#261157,#261158,#261159,#261160,#261161,#261162,#261163,
#261164,#261165,#261166,#261167,#261168,#261169,#261170,#261171,#261172,
#261173,#261174,#261175,#261176,#261177,#261178,#261179,#261180,#261181,
#261182,#261183,#261184,#261185,#261186,#261187,#261188,#261189,#261190,
#261191,#261192,#261193,#261194,#261195,#261196,#261197,#261198,#261199,
#261200,#261201,#261202,#261203,#261204,#261205,#261206,#261207,#261208,
#261209,#261210,#261211,#261212,#261213,#261214,#261215,#261216,#261217,
#261218,#261219,#261220,#261221,#261222),.UNSPECIFIED.,.F.,.F.,(4,3,3,3,
3,3,3,3,3,3,3,3,3,3,3,3,3,3,3,3,3,3,3,3,3,3,3,3,3,3,3,3,3,3,3,3,3,3,3,3,
3,3,3,3,3,3,3,3,3,3,3,3,3,3,3,3,3,3,3,3,3,3,3,3,3,3,3,3,3,3,3,3,3,3,3,4),
(0.517250288622702,0.523255252567395,0.529317273923346,0.532336217100087,
0.54742214558073,0.554965109821051,0.558736591941211,0.560984868363799,
0.562508074061372,0.575309787848133,0.587670338105941,0.59267993102266,
0.594690385794448,0.59645141314282,0.600222895262981,0.607765859503303,
0.61563385168986,0.622851787983946,0.626623270104107,0.630394752224268,
0.63793771646459,0.64603114658351,0.653023644945233,0.657541656586839,0.661717061888072,
0.665801492151527,0.668109573425877,0.680867615175072,0.68319550190652,
0.688004367601044,0.690738466146842,0.698281430387163,0.713367358867807,
0.722548733192488,0.72845328734845,0.741175990591504,0.753961138408387,
0.758625144309736,0.769291746524225,0.779988105774088,0.788797001271023,
0.796496519523186,0.804170797139037,0.811964278685929,0.818968858232309,
0.831626226508475,0.834054786712953,0.841597750953274,0.843483492013354,
0.844855917285564,0.845369233073435,0.849140715193595,0.857152162195407,
0.864226643674235,0.871769607914556,0.875275194327448,0.878806455714996,
0.879312572154876,0.887281929206424,0.894398500635516,0.901941464875837,
0.905712946995997,0.907623388041,0.909484429116157,0.921918691453167,0.924570357596798,
0.929478920092114,0.934567603084776,0.939344380756149,0.939656286077438,
0.954742214558079,0.96068040362499,0.966603908881514,0.969828143038719,
0.988792740999909,1.),.UNSPECIFIED.);
#5346=B_SPLINE_CURVE_WITH_KNOTS('',3,(#261226,#261227,#261228,#261229,#261230,
#261231,#261232,#261233,#261234,#261235,#261236,#261237,#261238,#261239,
#261240,#261241,#261242,#261243,#261244,#261245,#261246,#261247,#261248,
#261249,#261250,#261251,#261252,#261253,#261254,#261255,#261256,#261257,
#261258,#261259,#261260,#261261,#261262),.UNSPECIFIED.,.F.,.F.,(4,3,3,3,
3,3,3,3,3,3,3,3,4),(0.,0.0468962635573076,0.0985681948353279,0.120655574161669,
0.180983361242503,0.231914910914981,0.241311148323338,0.291000585436755,
0.346352184925574,0.361966722485007,0.422294509538762,0.471550853402632,
0.482622296592518),.UNSPECIFIED.);
#5347=B_SPLINE_CURVE_WITH_KNOTS('',3,(#261267,#261268,#261269,#261270,#261271,
#261272),.UNSPECIFIED.,.F.,.F.,(4,2,4),(-0.0139153924787358,-0.00694184678164755,
0.),.UNSPECIFIED.);
#5348=B_SPLINE_CURVE_WITH_KNOTS('',3,(#261275,#261276,#261277,#261278,#261279,
#261280,#261281,#261282,#261283,#261284,#261285,#261286,#261287,#261288,
#261289,#261290,#261291,#261292,#261293,#261294,#261295,#261296,#261297,
#261298,#261299,#261300,#261301,#261302,#261303,#261304,#261305,#261306,
#261307,#261308,#261309,#261310,#261311,#261312,#261313,#261314,#261315,
#261316,#261317),.UNSPECIFIED.,.F.,.F.,(4,3,3,3,3,3,3,3,3,3,3,3,3,3,4),
(0.499862670899252,0.507408441954982,0.514954213010712,0.530045755122171,
0.56022883934509,0.620595007790929,0.680961176236767,0.731927837407809,
0.741327344682605,0.790836072123878,0.801693513128444,0.862059681574282,
0.922425850020121,0.971634165151682,0.982792018465959),.UNSPECIFIED.);
#5349=B_SPLINE_CURVE_WITH_KNOTS('',3,(#261318,#261319,#261320,#261321,#261322,
#261323),.UNSPECIFIED.,.F.,.F.,(4,2,4),(0.482622296646676,0.491242483772964,
0.499862670899252),.UNSPECIFIED.);
#5350=B_SPLINE_CURVE_WITH_KNOTS('',3,(#261330,#261331,#261332,#261333,#261334,
#261335,#261336,#261337,#261338,#261339,#261340,#261341,#261342,#261343,
#261344,#261345,#261346,#261347,#261348,#261349,#261350,#261351,#261352,
#261353,#261354,#261355,#261356,#261357,#261358,#261359,#261360,#261361,
#261362,#261363,#261364,#261365,#261366,#261367,#261368,#261369,#261370,
#261371,#261372,#261373,#261374,#261375,#261376,#261377,#261378,#261379,
#261380,#261381,#261382,#261383,#261384,#261385,#261386,#261387,#261388,
#261389,#261390,#261391,#261392,#261393,#261394,#261395,#261396,#261397,
#261398,#261399,#261400,#261401,#261402,#261403,#261404,#261405,#261406,
#261407,#261408,#261409),.UNSPECIFIED.,.F.,.F.,(4,2,2,1,2,2,2,2,2,1,2,2,
2,2,2,2,2,2,1,2,2,2,2,2,2,1,2,2,2,2,2,2,2,2,2,2,2,2,2,2,2,4),(0.0173426649164943,
0.03242039763714,0.0474981303577856,0.0550369967181086,0.0588064298982699,
0.0625758630784312,0.0776535957990762,0.0927313285197211,0.0965007616998823,
0.100270194880043,0.107809061240366,0.122886793961012,0.130425660321335,
0.137964526681658,0.153042259402304,0.16811999212295,0.183197724843596,
0.190736591203919,0.198275457564241,0.213353190284887,0.228430923005532,
0.258586388446823,0.288741853888114,0.318897319329405,0.33397505205005,
0.341513918410373,0.343398635000453,0.345283351590534,0.349052784770696,
0.364130517491342,0.371669383851665,0.379208250211988,0.394285982932634,
0.401824849292957,0.405594282473119,0.409363715653281,0.424441448373927,
0.431980314734249,0.439519181094572,0.454596913815217,0.469674646535862,
0.499830111977151),.UNSPECIFIED.);
#5351=B_SPLINE_CURVE_WITH_KNOTS('',3,(#261494,#261495,#261496,#261497,#261498,
#261499,#261500,#261501,#261502,#261503,#261504,#261505,#261506,#261507,
#261508,#261509,#261510,#261511,#261512,#261513,#261514,#261515,#261516,
#261517,#261518,#261519,#261520,#261521,#261522,#261523,#261524,#261525,
#261526,#261527),.UNSPECIFIED.,.T.,.F.,(4,2,2,2,2,2,2,2,2,2,2,2,2,2,2,2,
4),(-0.765447565020067,-0.717607092096355,-0.669766619172642,-0.621926146468846,
-0.574085673765051,-0.526245201061255,-0.478404728357459,-0.430564255433746,
-0.382723782510034,-0.334883309586321,-0.287042836662609,-0.239202363958813,
-0.191361891255017,-0.143521418551221,-0.0956809458474253,-0.0478404729237126,
0.),.UNSPECIFIED.);
#5352=B_SPLINE_CURVE_WITH_KNOTS('',3,(#261531,#261532,#261533,#261534,#261535,
#261536,#261537,#261538,#261539,#261540,#261541,#261542,#261543,#261544,
#261545,#261546,#261547,#261548),.UNSPECIFIED.,.F.,.F.,(4,2,2,2,2,2,2,2,
4),(0.956809167700879,1.00464962597846,1.05249008425605,1.10033054274855,
1.14817100124105,1.19601145973356,1.24385191822606,1.29169237650364,1.33953283478123),
 .UNSPECIFIED.);
#5353=B_SPLINE_CURVE_WITH_KNOTS('',3,(#261549,#261550,#261551,#261552,#261553,
#261554,#261555,#261556,#261557,#261558,#261559,#261560,#261561,#261562,
#261563,#261564,#261565,#261566,#261567),.UNSPECIFIED.,.F.,.F.,(4,2,2,2,
3,2,2,2,4),(0.574085500620527,0.621925958898112,0.669766417175697,0.7176068756682,
0.765447334160703,0.813287792653206,0.861128251145709,0.908968709423294,
0.956809167700879),.UNSPECIFIED.);
#5354=B_SPLINE_CURVE_WITH_KNOTS('',3,(#261873,#261874,#261875,#261876,#261877,
#261878,#261879,#261880,#261881,#261882),.UNSPECIFIED.,.F.,.F.,(4,2,2,2,
4),(19.6371758899578,19.7291819054161,19.9154716265794,20.0518637703248,
20.1905913221304),.UNSPECIFIED.);
#5355=B_SPLINE_CURVE_WITH_KNOTS('',3,(#261888,#261889,#261890,#261891,#261892,
#261893,#261894,#261895,#261896,#261897,#261898,#261899,#261900,#261901,
#261902,#261903,#261904,#261905,#261906,#261907,#261908,#261909,#261910,
#261911,#261912,#261913,#261914,#261915,#261916,#261917,#261918,#261919,
#261920,#261921,#261922,#261923),.UNSPECIFIED.,.F.,.F.,(4,2,2,2,2,2,2,2,
2,2,2,2,2,2,2,2,2,4),(16.6532889927069,16.7775365014372,16.9626226669129,
17.1467233234454,17.331948216841,17.5158171192104,17.7011850850757,17.884830555016,
18.0703454741475,18.2537770495698,18.4394423104237,18.6226706701434,18.808489146925,
18.9915260123618,19.1775000503537,19.3603580661552,19.5464894746256,19.6371758899578),
 .UNSPECIFIED.);
#5356=B_SPLINE_CURVE_WITH_KNOTS('',3,(#261926,#261927,#261928,#261929,#261930,
#261931,#261932,#261933,#261934,#261935,#261936,#261937),.UNSPECIFIED.,
 .F.,.F.,(4,2,2,2,2,4),(9.99999997842682E-7,0.10581475344356,0.211369364467524,
0.394149985478841,0.581856914636482,0.656719561619648),.UNSPECIFIED.);
#5357=B_SPLINE_CURVE_WITH_KNOTS('',3,(#261942,#261943,#261944,#261945,#261946,
#261947,#261948,#261949,#261950,#261951,#261952,#261953,#261954,#261955,
#261956,#261957,#261958,#261959,#261960,#261961,#261962,#261963,#261964,
#261965,#261966,#261967,#261968,#261969,#261970,#261971,#261972,#261973,
#261974,#261975,#261976,#261977),.UNSPECIFIED.,.F.,.F.,(4,2,2,2,2,2,2,2,
2,2,2,2,2,2,2,2,2,4),(13.6684718789331,13.8194715122135,14.0036466813659,
14.1897487733689,14.3740161516353,14.5598650655264,14.7442311750837,14.9298255267918,
15.1142967841269,15.2996362197495,15.4842188879179,15.6693041664741,15.8540043062326,
16.0388373706964,16.223660791414,16.4082448250315,16.5931970363782,16.6532889927069),
 .UNSPECIFIED.);
#5358=B_SPLINE_CURVE_WITH_KNOTS('',3,(#261978,#261979,#261980,#261981,#261982,
#261983,#261984,#261985,#261986,#261987,#261988,#261989,#261990,#261991,
#261992,#261993,#261994,#261995,#261996,#261997,#261998,#261999,#262000,
#262001,#262002,#262003,#262004,#262005,#262006,#262007,#262008,#262009,
#262010,#262011,#262012,#262013),.UNSPECIFIED.,.F.,.F.,(4,2,2,2,2,2,2,2,
2,2,2,2,2,2,2,2,2,4),(0.656719561619648,0.764725887991887,0.952274080930713,
1.1352463285811,1.3226346599957,1.50572511626435,1.69295320251444,1.87617682495507,
2.06324476751678,2.24661625179435,2.43352466543164,2.61705847632778,2.80380850385605,
2.9875183338738,3.17411164750623,3.3580104164237,3.54444922709864,3.65228028819508),
 .UNSPECIFIED.);
#5359=B_SPLINE_CURVE_WITH_KNOTS('',3,(#262018,#262019,#262020,#262021,#262022,
#262023,#262024,#262025,#262026,#262027,#262028,#262029,#262030,#262031,
#262032,#262033,#262034,#262035,#262036,#262037,#262038,#262039,#262040,
#262041,#262042,#262043,#262044,#262045,#262046,#262047,#262048,#262049,
#262050,#262051,#262052,#262053),.UNSPECIFIED.,.F.,.F.,(4,2,2,2,2,2,2,2,
2,2,2,2,2,2,2,2,2,4),(10.6812382920827,10.851104857409,11.0347760974326,
11.2227618551089,11.4064741773505,11.5942433522979,11.7780027399581,11.9655491785976,
12.1493617836479,12.3366796007057,12.5205517225559,12.70763538643,12.8915734467528,
13.0784178707585,13.262428384412,13.4490290228049,13.6331185648837,13.6684718789331),
 .UNSPECIFIED.);
#5360=B_SPLINE_CURVE_WITH_KNOTS('',3,(#262054,#262055,#262056,#262057,#262058,
#262059,#262060,#262061,#262062,#262063,#262064,#262065,#262066,#262067,
#262068,#262069,#262070,#262071,#262072,#262073,#262074,#262075,#262076,
#262077,#262078,#262079,#262080,#262081,#262082,#262083,#262084,#262085,
#262086,#262087,#262088,#262089),.UNSPECIFIED.,.F.,.F.,(4,2,2,2,2,2,2,2,
2,2,2,2,2,2,2,2,2,4),(3.65228028819508,3.72854896313467,3.91483601545956,
4.0991477302083,4.28528628974196,4.4698198735951,4.65581370674877,4.84057784699934,
5.02643119406342,5.21143331699024,5.39715085899416,5.58239709631972,5.76798391659603,
5.95347909584702,6.13894063729285,6.32468829481463,6.51003031391758,6.64823144772819),
 .UNSPECIFIED.);
#5361=B_SPLINE_CURVE_WITH_KNOTS('',3,(#262094,#262095,#262096,#262097,#262098,
#262099,#262100,#262101,#262102,#262103,#262104,#262105,#262106,#262107,
#262108,#262109,#262110,#262111,#262112,#262113,#262114,#262115,#262116,
#262117,#262118,#262119,#262120,#262121,#262122,#262123,#262124,#262125,
#262126,#262127,#262128,#262129),.UNSPECIFIED.,.F.,.F.,(4,2,2,2,2,2,2,2,
2,2,2,2,2,2,2,2,2,4),(7.68984726224192,7.87165082930837,8.05518424630617,
8.24467155348332,8.42820570351524,8.61752739710676,8.80106654162163,8.99021654601221,
9.1737651724291,9.36273725215303,9.54630007523764,9.73508786455127,9.91866982592597,
10.1072668645547,10.2908731300591,10.479272905576,10.6629088601877,10.6812382920827),
 .UNSPECIFIED.);
#5362=B_SPLINE_CURVE_WITH_KNOTS('',3,(#262130,#262131,#262132,#262133,#262134,
#262135,#262136,#262137,#262138,#262139,#262140,#262141,#262142,#262143,
#262144,#262145,#262146,#262147,#262148,#262149,#262150,#262151,#262152,
#262153,#262154,#262155,#262156,#262157,#262158,#262159,#262160,#262161,
#262162,#262163,#262164,#262165),.UNSPECIFIED.,.F.,.F.,(4,2,2,2,2,2,2,2,
2,2,2,2,2,2,2,2,2,4),(6.64823144772819,6.69603272863731,6.88126124736131,
7.06751949288279,7.2526407494927,7.43915476174748,7.62417516159594,7.81094381907317,
7.99586988628593,8.17853506541196,8.3680551644229,8.55076973151589,8.74041126811349,
8.92318029343516,9.11294010138734,9.29576794379529,9.48564293206951,9.64577796424255),
 .UNSPECIFIED.);
#5363=B_SPLINE_CURVE_WITH_KNOTS('',3,(#262170,#262171,#262172,#262173,#262174,
#262175,#262176,#262177,#262178,#262179,#262180,#262181,#262182,#262183,
#262184,#262185,#262186,#262187,#262188,#262189,#262190,#262191,#262192,
#262193,#262194,#262195,#262196,#262197,#262198,#262199,#262200,#262201,
#262202,#262203,#262204,#262205),.UNSPECIFIED.,.F.,.F.,(4,2,2,2,2,2,2,2,
2,2,2,2,2,2,2,2,2,4),(4.69284812497761,4.87484108509642,5.06568438140767,
5.24914386949795,5.43990900710179,5.62329592544057,5.81398174998649,5.99729558403202,
6.18790085575909,6.37114111792534,6.56166450699332,6.74483074944173,6.93527083128246,
7.11836266102155,7.3087179117712,7.49173500832329,7.68200380040828,7.68984726224192),
 .UNSPECIFIED.);
#5364=B_SPLINE_CURVE_WITH_KNOTS('',3,(#262206,#262207,#262208,#262209,#262210,
#262211,#262212,#262213,#262214,#262215,#262216,#262217,#262218,#262219,
#262220,#262221,#262222,#262223,#262224,#262225,#262226,#262227,#262228,
#262229,#262230,#262231,#262232,#262233,#262234,#262235,#262236,#262237,
#262238,#262239,#262240,#262241),.UNSPECIFIED.,.F.,.F.,(4,2,2,2,2,2,2,2,
2,2,2,2,2,2,2,2,2,4),(9.64577796424255,9.66853329364696,9.85852045979922,
10.0414764425067,10.2315728834384,10.4145970462681,10.6047999665764,10.7878943819427,
10.9782011001008,11.1613674084466,11.3517753610505,11.5350148228858,11.7255215672028,
11.9088351120028,12.0994383270449,12.2828265986255,12.47352408496,12.6469505891598),
 .UNSPECIFIED.);
#5365=B_SPLINE_CURVE_WITH_KNOTS('',3,(#262246,#262247,#262248,#262249,#262250,
#262251,#262252,#262253,#262254,#262255,#262256,#262257,#262258,#262259,
#262260,#262261,#262262,#262263,#262264,#262265,#262266,#262267,#262268,
#262269,#262270,#262271,#262272,#262273,#262274,#262275,#262276,#262277,
#262278,#262279,#262280,#262281,#262282,#262283),.UNSPECIFIED.,.F.,.F.,
(4,2,2,2,2,2,2,2,2,2,2,2,2,2,2,2,2,2,4),(1.69140295334555,1.6939489277295,
1.87761272004276,2.06833630149064,2.25202774081888,2.44286910038617,2.62659054726916,
2.81754600595523,3.00129966734393,3.19236576281363,3.37615370027557,3.56729963547581,
3.75104405717415,3.9421156884852,4.12578967937756,4.3167861485705,4.5003891765768,
4.69130955801646,4.69284812497761),.UNSPECIFIED.);
#5366=B_SPLINE_CURVE_WITH_KNOTS('',3,(#262284,#262285,#262286,#262287,#262288,
#262289,#262290,#262291,#262292,#262293,#262294,#262295,#262296,#262297,
#262298,#262299,#262300,#262301,#262302,#262303,#262304,#262305,#262306,
#262307,#262308,#262309,#262310,#262311,#262312,#262313,#262314,#262315,
#262316,#262317,#262318,#262319),.UNSPECIFIED.,.F.,.F.,(4,2,2,2,2,2,2,2,
2,2,2,2,2,2,2,2,2,4),(12.6469505891598,12.6569874831093,12.8477771616045,
13.0313158798829,13.2221957895684,13.4058098493005,13.5967781445068,13.7804674250698,
13.9715223719929,14.1552866375716,14.3464266103928,14.5302655334145,14.721489010089,
14.9054021915795,15.0967077493918,15.2806947365115,15.4720810474833,15.6534010530854),
 .UNSPECIFIED.);
#5367=B_SPLINE_CURVE_WITH_KNOTS('',3,(#262326,#262327,#262328,#262329,#262330,
#262331,#262332,#262333,#262334,#262335,#262336,#262337,#262338,#262339,
#262340,#262341,#262342,#262343,#262344,#262345,#262346,#262347),
 .UNSPECIFIED.,.F.,.F.,(4,2,2,2,2,2,2,2,2,2,4),(1.0000000306154E-6,0.0999528028591011,
0.19788302817369,0.38146309163929,0.571674110669096,0.755270677145627,0.945616475624153,
1.12923260286766,1.31970857888015,1.50334713803867,1.69140295334555),
 .UNSPECIFIED.);
#5368=B_SPLINE_CURVE_WITH_KNOTS('',3,(#262348,#262349,#262350,#262351,#262352,
#262353,#262354,#262355,#262356,#262357,#262358,#262359,#262360,#262361,
#262362,#262363,#262364,#262365,#262366,#262367,#262368,#262369,#262370,
#262371,#262372,#262373,#262374,#262375,#262376,#262377,#262378,#262379,
#262380,#262381,#262382,#262383,#262384,#262385),.UNSPECIFIED.,.F.,.F.,
(4,2,2,2,2,2,2,2,2,2,2,2,2,2,2,2,2,2,4),(15.6534010530854,15.6561413485049,
15.8476071747258,16.031740271715,16.2232844606574,16.4074898201077,16.5991112999749,
16.7833883816353,16.9750861567836,17.1594344209024,17.3512075673696,17.5356002898847,
17.7273598918852,17.9117164451164,18.103368086355,18.2876904108166,18.4792308121127,
18.6635209866941,18.6649773663315),.UNSPECIFIED.);
#5369=B_SPLINE_CURVE_WITH_KNOTS('',3,(#262406,#262407,#262408,#262409,#262410,
#262411,#262412,#262413,#262414,#262415,#262416,#262417,#262418,#262419,
#262420,#262421,#262422,#262423,#262424,#262425),.UNSPECIFIED.,.F.,.F.,
(4,2,2,2,2,2,2,2,2,4),(18.6649773663315,18.8549465390401,19.0392066732075,
19.2305137878141,19.4147463775256,19.605931123255,19.7901387116017,19.9811969260739,
20.1223735917246,20.2610225738873),.UNSPECIFIED.);
#5370=B_SPLINE_CURVE_WITH_KNOTS('',3,(#263400,#263401,#263402,#263403,#263404,
#263405,#263406,#263407,#263408,#263409),.UNSPECIFIED.,.F.,.F.,(4,2,2,2,
4),(19.6371758899503,19.7291819054085,19.9154716265718,20.0518637703173,
20.1905913221229),.UNSPECIFIED.);
#5371=B_SPLINE_CURVE_WITH_KNOTS('',3,(#263415,#263416,#263417,#263418,#263419,
#263420,#263421,#263422,#263423,#263424,#263425,#263426,#263427,#263428,
#263429,#263430,#263431,#263432,#263433,#263434,#263435,#263436,#263437,
#263438,#263439,#263440,#263441,#263442,#263443,#263444,#263445,#263446,
#263447,#263448,#263449,#263450),.UNSPECIFIED.,.F.,.F.,(4,2,2,2,2,2,2,2,
2,2,2,2,2,2,2,2,2,4),(16.6532889927,16.7775365014302,16.9626226669059,17.1467233234384,
17.3319482168339,17.5158171192032,17.7011850850685,17.8848305550088,18.0703454741403,
18.2537770495626,18.4394423104164,18.6226706701361,18.8084891469176,18.9915260123544,
19.1775000503463,19.3603580661478,19.5464894746181,19.6371758899503),
 .UNSPECIFIED.);
#5372=B_SPLINE_CURVE_WITH_KNOTS('',3,(#263453,#263454,#263455,#263456,#263457,
#263458,#263459,#263460,#263461,#263462,#263463,#263464),.UNSPECIFIED.,
 .F.,.F.,(4,2,2,2,2,4),(9.99999998777405E-7,0.105814753443105,0.211369364466581,
0.3941499854778,0.581856914635303,0.656719561619345),.UNSPECIFIED.);
#5373=B_SPLINE_CURVE_WITH_KNOTS('',3,(#263469,#263470,#263471,#263472,#263473,
#263474,#263475,#263476,#263477,#263478,#263479,#263480,#263481,#263482,
#263483,#263484,#263485,#263486,#263487,#263488,#263489,#263490,#263491,
#263492,#263493,#263494,#263495,#263496,#263497,#263498,#263499,#263500,
#263501,#263502,#263503,#263504),.UNSPECIFIED.,.F.,.F.,(4,2,2,2,2,2,2,2,
2,2,2,2,2,2,2,2,2,4),(13.6684718789269,13.8194715122071,14.0036466813595,
14.1897487733625,14.3740161516288,14.5598650655198,14.7442311750771,14.9298255267851,
15.1142967841201,15.2996362197427,15.4842188879111,15.6693041664674,15.8540043062258,
16.0388373706896,16.2236607914072,16.4082448250246,16.5931970363712,16.6532889927),
 .UNSPECIFIED.);
#5374=B_SPLINE_CURVE_WITH_KNOTS('',3,(#263505,#263506,#263507,#263508,#263509,
#263510,#263511,#263512,#263513,#263514,#263515,#263516,#263517,#263518,
#263519,#263520,#263521,#263522,#263523,#263524,#263525,#263526,#263527,
#263528,#263529,#263530,#263531,#263532,#263533,#263534,#263535,#263536,
#263537,#263538,#263539,#263540),.UNSPECIFIED.,.F.,.F.,(4,2,2,2,2,2,2,2,
2,2,2,2,2,2,2,2,2,4),(0.656719561619345,0.764725887990629,0.95227408092929,
1.13524632857959,1.32263465999408,1.50572511626269,1.69295320251266,1.87617682495327,
2.06324476751485,2.24661625179239,2.43352466542956,2.61705847632565,2.80380850385381,
2.98751833387153,3.17411164750387,3.35801041642132,3.54444922709616,3.65228028819351),
 .UNSPECIFIED.);
#5375=B_SPLINE_CURVE_WITH_KNOTS('',3,(#263545,#263546,#263547,#263548,#263549,
#263550,#263551,#263552,#263553,#263554,#263555,#263556,#263557,#263558,
#263559,#263560,#263561,#263562,#263563,#263564,#263565,#263566,#263567,
#263568,#263569,#263570,#263571,#263572,#263573,#263574,#263575,#263576,
#263577,#263578,#263579,#263580),.UNSPECIFIED.,.F.,.F.,(4,2,2,2,2,2,2,2,
2,2,2,2,2,2,2,2,2,4),(10.6812382920774,10.8511048574036,11.0347760974271,
11.2227618551033,11.4064741773449,11.5942433522923,11.7780027399524,11.9655491785918,
12.1493617836421,12.3366796006998,12.5205517225499,12.7076353864239,12.8915734467467,
13.0784178707524,13.2624283844058,13.4490290227987,13.6331185648774,13.6684718789269),
 .UNSPECIFIED.);
#5376=B_SPLINE_CURVE_WITH_KNOTS('',3,(#263581,#263582,#263583,#263584,#263585,
#263586,#263587,#263588,#263589,#263590,#263591,#263592,#263593,#263594,
#263595,#263596,#263597,#263598,#263599,#263600,#263601,#263602,#263603,
#263604,#263605,#263606,#263607,#263608,#263609,#263610,#263611,#263612,
#263613,#263614,#263615,#263616),.UNSPECIFIED.,.F.,.F.,(4,2,2,2,2,2,2,2,
2,2,2,2,2,2,2,2,2,4),(3.65228028819351,3.72854896313221,3.91483601545701,
4.09914773020572,4.28528628973924,4.46981987359233,4.65581370674584,4.84057784699636,
5.0264311940603,5.21143331698707,5.39715085899084,5.58239709631633,5.76798391659248,
5.95347909584341,6.13894063728909,6.32468829481084,6.51003031391372,6.64823144772506),
 .UNSPECIFIED.);
#5377=B_SPLINE_CURVE_WITH_KNOTS('',3,(#263621,#263622,#263623,#263624,#263625,
#263626,#263627,#263628,#263629,#263630,#263631,#263632,#263633,#263634,
#263635,#263636,#263637,#263638,#263639,#263640,#263641,#263642,#263643,
#263644,#263645,#263646,#263647,#263648,#263649,#263650,#263651,#263652,
#263653,#263654,#263655,#263656),.UNSPECIFIED.,.F.,.F.,(4,2,2,2,2,2,2,2,
2,2,2,2,2,2,2,2,2,4),(7.689847262238,7.87165082930434,8.05518424630204,
8.24467155347909,8.42820570351091,8.61752739710234,8.8010665416171,8.99021654600758,
9.1737651724244,9.36273725214825,9.5463000752328,9.73508786454633,9.91866982592094,
10.1072668645495,10.2908731300539,10.4792729055708,10.6629088601823,10.6812382920774),
 .UNSPECIFIED.);
#5378=B_SPLINE_CURVE_WITH_KNOTS('',3,(#263657,#263658,#263659,#263660,#263661,
#263662,#263663,#263664,#263665,#263666,#263667,#263668,#263669,#263670,
#263671,#263672,#263673,#263674,#263675,#263676,#263677,#263678,#263679,
#263680,#263681,#263682,#263683,#263684,#263685,#263686,#263687,#263688,
#263689,#263690,#263691,#263692),.UNSPECIFIED.,.F.,.F.,(4,2,2,2,2,2,2,2,
2,2,2,2,2,2,2,2,2,4),(6.64823144772506,6.69603272863345,6.88126124735736,
7.06751949287885,7.25264074948867,7.43915476174343,7.6241751615918,7.81094381906902,
7.99586988628166,8.17853506540754,8.36805516441837,8.55076973151126,8.74041126810875,
8.92318029343032,9.11294010138241,9.29576794379026,9.48564293206439,9.64577796423785),
 .UNSPECIFIED.);
#5379=B_SPLINE_CURVE_WITH_KNOTS('',3,(#263697,#263698,#263699,#263700,#263701,
#263702,#263703,#263704,#263705,#263706,#263707,#263708,#263709,#263710,
#263711,#263712,#263713,#263714,#263715,#263716,#263717,#263718,#263719,
#263720,#263721,#263722,#263723,#263724,#263725,#263726,#263727,#263728,
#263729,#263730,#263731,#263732),.UNSPECIFIED.,.F.,.F.,(4,2,2,2,2,2,2,2,
2,2,2,2,2,2,2,2,2,4),(4.69284812497508,4.87484108509382,5.06568438140499,
5.2491438694952,5.43990900709896,5.62329592543766,5.8139817499835,5.99729558402895,
6.18790085575593,6.37114111792207,6.56166450698997,6.74483074943831,6.93527083127893,
7.11836266101793,7.30871791176746,7.49173500831945,7.68200380040434,7.689847262238),
 .UNSPECIFIED.);
#5380=B_SPLINE_CURVE_WITH_KNOTS('',3,(#263733,#263734,#263735,#263736,#263737,
#263738,#263739,#263740,#263741,#263742,#263743,#263744,#263745,#263746,
#263747,#263748,#263749,#263750,#263751,#263752,#263753,#263754,#263755,
#263756,#263757,#263758,#263759,#263760,#263761,#263762,#263763,#263764,
#263765,#263766,#263767,#263768),.UNSPECIFIED.,.F.,.F.,(4,2,2,2,2,2,2,2,
2,2,2,2,2,2,2,2,2,4),(9.64577796423785,9.66853329364174,9.8585204597939,
10.0414764425013,10.2315728834329,10.4145970462625,10.6047999665707,10.7878943819369,
10.9782011000949,11.1613674084406,11.3517753610445,11.5350148228797,11.7255215671966,
11.9088351119965,12.0994383270385,12.2828265986191,12.4735240849535,12.6469505891534),
 .UNSPECIFIED.);
#5381=B_SPLINE_CURVE_WITH_KNOTS('',3,(#263773,#263774,#263775,#263776,#263777,
#263778,#263779,#263780,#263781,#263782,#263783,#263784,#263785,#263786,
#263787,#263788,#263789,#263790,#263791,#263792,#263793,#263794,#263795,
#263796,#263797,#263798,#263799,#263800,#263801,#263802,#263803,#263804,
#263805,#263806,#263807,#263808,#263809,#263810),.UNSPECIFIED.,.F.,.F.,
(4,2,2,2,2,2,2,2,2,2,2,2,2,2,2,2,2,2,4),(1.69140295334456,1.6939489277285,
1.87761272004166,2.06833630148944,2.25202774081757,2.44286910038474,2.62659054726762,
2.81754600595354,3.00129966734211,3.19236576281171,3.37615370027357,3.56729963547373,
3.75104405717199,3.94211568848297,4.12578967937525,4.31678614856811,4.50038917657433,
4.69130955801392,4.69284812497508),.UNSPECIFIED.);
#5382=B_SPLINE_CURVE_WITH_KNOTS('',3,(#263811,#263812,#263813,#263814,#263815,
#263816,#263817,#263818,#263819,#263820,#263821,#263822,#263823,#263824,
#263825,#263826,#263827,#263828,#263829,#263830,#263831,#263832,#263833,
#263834,#263835,#263836,#263837,#263838,#263839,#263840,#263841,#263842,
#263843,#263844,#263845,#263846),.UNSPECIFIED.,.F.,.F.,(4,2,2,2,2,2,2,2,
2,2,2,2,2,2,2,2,2,4),(12.6469505891534,12.6569874831027,12.8477771615977,
13.031315879876,13.2221957895613,13.4058098492933,13.5967781444994,13.7804674250622,
13.9715223719852,14.1552866375637,14.3464266103848,14.5302655334064,14.7214890100807,
14.9054021915711,15.0967077493834,15.2806947365029,15.4720810474746,15.6534010530768),
 .UNSPECIFIED.);
#5383=B_SPLINE_CURVE_WITH_KNOTS('',3,(#263853,#263854,#263855,#263856,#263857,
#263858,#263859,#263860,#263861,#263862,#263863,#263864,#263865,#263866,
#263867,#263868,#263869,#263870,#263871,#263872,#263873,#263874),
 .UNSPECIFIED.,.F.,.F.,(4,2,2,2,2,2,2,2,2,2,4),(9.99999998962388E-7,0.0999528028590244,
0.197883028173547,0.381463091639027,0.571674110668726,0.755270677145161,
0.945616475623583,1.12923260286698,1.31970857887937,1.50334713803778,1.69140295334456),
 .UNSPECIFIED.);
#5384=B_SPLINE_CURVE_WITH_KNOTS('',3,(#263875,#263876,#263877,#263878,#263879,
#263880,#263881,#263882,#263883,#263884,#263885,#263886,#263887,#263888,
#263889,#263890,#263891,#263892,#263893,#263894,#263895,#263896,#263897,
#263898,#263899,#263900,#263901,#263902,#263903,#263904,#263905,#263906,
#263907,#263908,#263909,#263910,#263911,#263912),.UNSPECIFIED.,.F.,.F.,
(4,2,2,2,2,2,2,2,2,2,2,2,2,2,2,2,2,2,4),(15.6534010530768,15.6561413484961,
15.8476071747169,16.031740271706,16.2232844606483,16.4074898200985,16.5991112999656,
16.7833883816259,16.975086156774,17.1594344208927,17.3512075673597,17.5356002898748,
17.7273598918751,17.9117164451062,18.1033680863446,18.2876904108061,18.479230812102,
18.6635209866833,18.6649773663208),.UNSPECIFIED.);
#5385=B_SPLINE_CURVE_WITH_KNOTS('',3,(#263933,#263934,#263935,#263936,#263937,
#263938,#263939,#263940,#263941,#263942,#263943,#263944,#263945,#263946,
#263947,#263948,#263949,#263950,#263951,#263952),.UNSPECIFIED.,.F.,.F.,
(4,2,2,2,2,2,2,2,2,4),(18.6649773663208,18.8549465390291,19.0392066731962,
19.2305137878026,19.414746377514,19.6059311232431,19.7901387115896,19.9811969260615,
20.1223735917122,20.2610225738747),.UNSPECIFIED.);
#5386=B_SPLINE_CURVE_WITH_KNOTS('',3,(#264727,#264728,#264729,#264730,#264731,
#264732,#264733,#264734,#264735,#264736,#264737,#264738,#264739,#264740,
#264741,#264742,#264743,#264744),.UNSPECIFIED.,.F.,.F.,(4,2,2,2,2,2,2,2,
4),(-2.15416629289221,-1.97465268640277,-1.79513907991332,-1.61562497092073,
-1.43611086192814,-1.25659675293555,-1.07708264394295,-0.897569037453512,
-0.718055430964069),.UNSPECIFIED.);
#5387=B_SPLINE_CURVE_WITH_KNOTS('',3,(#264746,#264747,#264748,#264749,#264750,
#264751,#264752,#264753,#264754,#264755,#264756,#264757,#264758,#264759,
#264760,#264761,#264762,#264763,#264764),.UNSPECIFIED.,.F.,.F.,(4,2,2,2,
3,2,2,2,4),(-0.718055430964069,-0.538541824474627,-0.359028217985184,-0.179514108992592,
0.,0.179514108992592,0.359028217985184,0.538541824474627,0.71805543096407),
 .UNSPECIFIED.);
#5388=B_SPLINE_CURVE_WITH_KNOTS('',3,(#264767,#264768,#264769,#264770,#264771,
#264772,#264773,#264774,#264775,#264776,#264777,#264778,#264779,#264780,
#264781,#264782,#264783,#264784,#264785),.UNSPECIFIED.,.F.,.F.,(4,2,2,2,
3,2,2,2,4),(2.15416629289221,2.33367989938165,2.51319350587109,2.69270761486369,
2.87222172385628,3.05173583284887,3.23124994184146,3.4107635483309,3.59027715482035),
 .UNSPECIFIED.);
#5389=B_SPLINE_CURVE_WITH_KNOTS('',3,(#264786,#264787,#264788,#264789,#264790,
#264791,#264792,#264793,#264794,#264795,#264796,#264797,#264798,#264799,
#264800,#264801,#264802,#264803),.UNSPECIFIED.,.F.,.F.,(4,2,2,2,2,2,2,2,
4),(3.59027715482035,3.76979076130979,3.94930436779923,4.12881847679182,
4.30833258578442,4.48784669477701,4.6673608037696,4.84687441025904,5.02638801674849),
 .UNSPECIFIED.);
#5390=B_SPLINE_CURVE_WITH_KNOTS('',3,(#264807,#264808,#264809,#264810,#264811,
#264812,#264813,#264814,#264815,#264816,#264817,#264818,#264819,#264820,
#264821,#264822,#264823,#264824,#264825,#264826,#264827,#264828,#264829,
#264830,#264831,#264832,#264833,#264834,#264835,#264836,#264837,#264838,
#264839,#264840),.UNSPECIFIED.,.T.,.F.,(4,2,2,2,2,2,2,2,2,2,2,2,2,2,2,2,
4),(0.,0.179580636707928,0.359161273415856,0.538740676948295,0.718320080480733,
0.897899484013172,1.07747888754561,1.25705952425354,1.43664016096147,1.61622079766939,
1.79580143437732,1.97538083790976,2.1549602414422,2.33453964497464,2.51411904850708,
2.693699685215,2.87328032192293),.UNSPECIFIED.);
#5391=B_SPLINE_CURVE_WITH_KNOTS('',3,(#264845,#264846,#264847,#264848,#264849,
#264850,#264851,#264852,#264853,#264854,#264855,#264856,#264857,#264858,
#264859,#264860,#264861,#264862,#264863),.UNSPECIFIED.,.F.,.F.,(4,2,2,2,
3,2,2,2,4),(2.1549602414422,2.33453964497464,2.51411904850708,2.693699685215,
2.87328032192293,3.05286095863086,3.23244159533879,3.41202099887123,3.59160040240367),
 .UNSPECIFIED.);
#5392=B_SPLINE_CURVE_WITH_KNOTS('',3,(#264864,#264865,#264866,#264867,#264868,
#264869,#264870,#264871,#264872,#264873,#264874,#264875,#264876,#264877,
#264878,#264879,#264880,#264881),.UNSPECIFIED.,.F.,.F.,(4,2,2,2,2,2,2,2,
4),(0.718320080480733,0.897899484013172,1.07747888754561,1.25705952425354,
1.43664016096147,1.61622079766939,1.79580143437732,1.97538083790976,2.1549602414422),
 .UNSPECIFIED.);
#5462=SHAPE_REPRESENTATION_RELATIONSHIP('SRR','None',#276490,#5468);
#5468=ADVANCED_BREP_SHAPE_REPRESENTATION('',(#5504,#5505,#5506,#5507,#5508,
#5509,#5510,#5511,#5512,#5513,#5514,#5515,#5516,#5517,#5518,#5519,#5520,
#5521,#5522,#5523,#5524),#276458);
#5475=STYLED_ITEM('',(#276529),#5504);
#5476=STYLED_ITEM('',(#276529),#5505);
#5477=STYLED_ITEM('',(#276529),#5506);
#5478=STYLED_ITEM('',(#276529),#5507);
#5479=STYLED_ITEM('',(#276529),#5508);
#5480=STYLED_ITEM('',(#276529),#5509);
#5481=STYLED_ITEM('',(#276529),#5510);
#5482=STYLED_ITEM('',(#276529),#5511);
#5483=STYLED_ITEM('',(#276529),#5512);
#5484=STYLED_ITEM('',(#276529),#5513);
#5485=STYLED_ITEM('',(#276529),#5514);
#5486=STYLED_ITEM('',(#276529),#5515);
#5487=STYLED_ITEM('',(#276529),#5516);
#5488=STYLED_ITEM('',(#276529),#5517);
#5489=STYLED_ITEM('',(#276529),#5518);
#5490=STYLED_ITEM('',(#276529),#5519);
#5491=STYLED_ITEM('',(#276529),#5520);
#5492=STYLED_ITEM('',(#276529),#5521);
#5493=STYLED_ITEM('',(#276529),#5522);
#5494=STYLED_ITEM('',(#276529),#5523);
#5495=STYLED_ITEM('',(#276529),#5524);
#5504=MANIFOLD_SOLID_BREP('Body1',#98700);
#5505=MANIFOLD_SOLID_BREP('Body2',#98701);
#5506=MANIFOLD_SOLID_BREP('Body3',#98702);
#5507=MANIFOLD_SOLID_BREP('Body4',#98703);
#5508=MANIFOLD_SOLID_BREP('Body5',#98704);
#5509=MANIFOLD_SOLID_BREP('Body6',#98705);
#5510=MANIFOLD_SOLID_BREP('Body7',#98706);
#5511=MANIFOLD_SOLID_BREP('Body8',#98707);
#5512=MANIFOLD_SOLID_BREP('Body9',#98708);
#5513=MANIFOLD_SOLID_BREP('Body10',#98709);
#5514=MANIFOLD_SOLID_BREP('Body11',#98710);
#5515=MANIFOLD_SOLID_BREP('Body12',#98711);
#5516=MANIFOLD_SOLID_BREP('Body13',#98712);
#5517=MANIFOLD_SOLID_BREP('Body14',#98713);
#5518=MANIFOLD_SOLID_BREP('Body15',#98714);
#5519=MANIFOLD_SOLID_BREP('Body16',#98715);
#5520=MANIFOLD_SOLID_BREP('Body17',#98716);
#5521=MANIFOLD_SOLID_BREP('Body18',#98717);
#5522=MANIFOLD_SOLID_BREP('Body19',#98718);
#5523=MANIFOLD_SOLID_BREP('Body20',#98719);
#5524=MANIFOLD_SOLID_BREP('Body21',#98720);
#5535=TOROIDAL_SURFACE('',#98940,4.30674336537535,1.57226);
#5536=TOROIDAL_SURFACE('',#98962,2.71842830011631,0.635000000000008);
#5537=TOROIDAL_SURFACE('',#98969,2.1119189867422,0.317500000000003);
#5538=TOROIDAL_SURFACE('',#99037,50.254,0.254);
#5539=TOROIDAL_SURFACE('',#99042,51.016,0.254);
#5540=TOROIDAL_SURFACE('',#99053,56.621,0.254);
#5541=TOROIDAL_SURFACE('',#99058,55.859,0.254);
#5542=TOROIDAL_SURFACE('',#99077,59.0285554514622,0.127);
#5543=TOROIDAL_SURFACE('',#99082,62.8464445485378,0.127);
#5544=TOROIDAL_SURFACE('',#99087,59.0285554514622,0.127);
#5545=TOROIDAL_SURFACE('',#99092,62.8464445485378,0.127);
#5546=TOROIDAL_SURFACE('',#99098,58.2189663438286,0.635);
#5547=TOROIDAL_SURFACE('',#99103,58.3085779254084,0.635);
#5548=TOROIDAL_SURFACE('',#99107,63.5664220745916,0.635);
#5549=TOROIDAL_SURFACE('',#99112,63.6560336561714,0.635);
#5550=TOROIDAL_SURFACE('',#99381,60.0045305169095,0.635);
#5551=TOROIDAL_SURFACE('',#99384,61.8704694830905,0.635);
#5552=TOROIDAL_SURFACE('',#99387,61.0131030316259,0.254);
#5553=TOROIDAL_SURFACE('',#99390,60.8618969683742,0.254);
#5554=TOROIDAL_SURFACE('',#99410,60.0045305169095,0.635);
#5555=TOROIDAL_SURFACE('',#99413,61.8704694830905,0.635);
#5556=TOROIDAL_SURFACE('',#99416,61.0131030316259,0.254);
#5557=TOROIDAL_SURFACE('',#99419,60.8618969683742,0.254);
#5558=TOROIDAL_SURFACE('',#99439,60.0045305169095,0.635);
#5559=TOROIDAL_SURFACE('',#99442,61.8704694830905,0.635);
#5560=TOROIDAL_SURFACE('',#99445,61.0131030316259,0.254);
#5561=TOROIDAL_SURFACE('',#99448,60.8618969683742,0.254);
#5562=TOROIDAL_SURFACE('',#99468,60.0045305169095,0.635);
#5563=TOROIDAL_SURFACE('',#99471,61.8704694830905,0.635);
#5564=TOROIDAL_SURFACE('',#99474,61.0131030316259,0.254);
#5565=TOROIDAL_SURFACE('',#99477,60.8618969683742,0.254);
#5566=TOROIDAL_SURFACE('',#99497,60.0045305169095,0.635);
#5567=TOROIDAL_SURFACE('',#99500,61.8704694830905,0.635);
#5568=TOROIDAL_SURFACE('',#99503,61.0131030316259,0.254);
#5569=TOROIDAL_SURFACE('',#99506,60.8618969683742,0.254);
#5570=TOROIDAL_SURFACE('',#99526,60.0045305169095,0.635);
#5571=TOROIDAL_SURFACE('',#99529,61.8704694830905,0.635);
#5572=TOROIDAL_SURFACE('',#99532,61.0131030316259,0.254);
#5573=TOROIDAL_SURFACE('',#99535,60.8618969683742,0.254);
#5574=TOROIDAL_SURFACE('',#99555,60.0045305169095,0.635);
#5575=TOROIDAL_SURFACE('',#99558,61.8704694830905,0.635);
#5576=TOROIDAL_SURFACE('',#99561,61.0131030316259,0.254);
#5577=TOROIDAL_SURFACE('',#99564,60.8618969683742,0.254);
#5578=TOROIDAL_SURFACE('',#99584,60.0045305169095,0.635);
#5579=TOROIDAL_SURFACE('',#99587,61.8704694830905,0.635);
#5580=TOROIDAL_SURFACE('',#99590,61.0131030316259,0.254);
#5581=TOROIDAL_SURFACE('',#99593,60.8618969683742,0.254);
#5582=TOROIDAL_SURFACE('',#99613,60.0045305169095,0.635);
#5583=TOROIDAL_SURFACE('',#99616,61.8704694830905,0.635);
#5584=TOROIDAL_SURFACE('',#99619,61.0131030316259,0.254);
#5585=TOROIDAL_SURFACE('',#99622,60.8618969683742,0.254);
#5586=TOROIDAL_SURFACE('',#99642,60.0045305169095,0.635);
#5587=TOROIDAL_SURFACE('',#99645,61.8704694830905,0.635);
#5588=TOROIDAL_SURFACE('',#99648,61.0131030316259,0.254);
#5589=TOROIDAL_SURFACE('',#99651,60.8618969683742,0.254);
#5590=TOROIDAL_SURFACE('',#99671,60.0045305169095,0.635);
#5591=TOROIDAL_SURFACE('',#99674,61.8704694830905,0.635);
#5592=TOROIDAL_SURFACE('',#99677,61.0131030316259,0.254);
#5593=TOROIDAL_SURFACE('',#99680,60.8618969683742,0.254);
#5594=TOROIDAL_SURFACE('',#99700,60.0045305169095,0.635);
#5595=TOROIDAL_SURFACE('',#99703,61.8704694830905,0.635);
#5596=TOROIDAL_SURFACE('',#99706,61.0131030316259,0.254);
#5597=TOROIDAL_SURFACE('',#99709,60.8618969683742,0.254);
#5598=TOROIDAL_SURFACE('',#99729,60.0045305169095,0.635);
#5599=TOROIDAL_SURFACE('',#99732,61.8704694830905,0.635);
#5600=TOROIDAL_SURFACE('',#99735,61.0131030316259,0.254);
#5601=TOROIDAL_SURFACE('',#99738,60.8618969683742,0.254);
#5602=TOROIDAL_SURFACE('',#99758,60.0045305169095,0.635);
#5603=TOROIDAL_SURFACE('',#99761,61.8704694830905,0.635);
#5604=TOROIDAL_SURFACE('',#99764,61.0131030316259,0.254);
#5605=TOROIDAL_SURFACE('',#99767,60.8618969683742,0.254);
#5606=TOROIDAL_SURFACE('',#99787,60.0045305169095,0.635);
#5607=TOROIDAL_SURFACE('',#99790,61.8704694830905,0.635);
#5608=TOROIDAL_SURFACE('',#99793,61.0131030316259,0.254);
#5609=TOROIDAL_SURFACE('',#99796,60.8618969683742,0.254);
#5610=TOROIDAL_SURFACE('',#99816,60.0045305169095,0.635);
#5611=TOROIDAL_SURFACE('',#99819,61.8704694830905,0.635);
#5612=TOROIDAL_SURFACE('',#99822,61.0131030316259,0.254);
#5613=TOROIDAL_SURFACE('',#99825,60.8618969683742,0.254);
#5614=TOROIDAL_SURFACE('',#99845,60.0045305169095,0.635);
#5615=TOROIDAL_SURFACE('',#99848,61.8704694830905,0.635);
#5616=TOROIDAL_SURFACE('',#99851,61.0131030316259,0.254);
#5617=TOROIDAL_SURFACE('',#99854,60.8618969683742,0.254);
#5618=TOROIDAL_SURFACE('',#99874,60.0045305169095,0.635);
#5619=TOROIDAL_SURFACE('',#99877,61.8704694830905,0.635);
#5620=TOROIDAL_SURFACE('',#99880,61.0131030316259,0.254);
#5621=TOROIDAL_SURFACE('',#99883,60.8618969683742,0.254);
#5622=TOROIDAL_SURFACE('',#99903,60.0045305169095,0.635);
#5623=TOROIDAL_SURFACE('',#99906,61.8704694830905,0.635);
#5624=TOROIDAL_SURFACE('',#99909,61.0131030316259,0.254);
#5625=TOROIDAL_SURFACE('',#99912,60.8618969683742,0.254);
#5626=TOROIDAL_SURFACE('',#99932,60.0045305169095,0.635);
#5627=TOROIDAL_SURFACE('',#99935,61.8704694830905,0.635);
#5628=TOROIDAL_SURFACE('',#99938,61.0131030316259,0.254);
#5629=TOROIDAL_SURFACE('',#99941,60.8618969683742,0.254);
#5630=TOROIDAL_SURFACE('',#99961,60.0045305169095,0.635);
#5631=TOROIDAL_SURFACE('',#99964,61.8704694830905,0.635);
#5632=TOROIDAL_SURFACE('',#99967,61.0131030316259,0.254);
#5633=TOROIDAL_SURFACE('',#99970,60.8618969683742,0.254);
#5634=TOROIDAL_SURFACE('',#99990,60.0045305169095,0.635);
#5635=TOROIDAL_SURFACE('',#99993,61.8704694830905,0.635);
#5636=TOROIDAL_SURFACE('',#99996,61.0131030316259,0.254);
#5637=TOROIDAL_SURFACE('',#99999,60.8618969683742,0.254);
#5638=TOROIDAL_SURFACE('',#100019,60.0045305169095,0.635);
#5639=TOROIDAL_SURFACE('',#100022,61.8704694830905,0.635);
#5640=TOROIDAL_SURFACE('',#100025,61.0131030316259,0.254);
#5641=TOROIDAL_SURFACE('',#100028,60.8618969683742,0.254);
#5642=TOROIDAL_SURFACE('',#100048,60.0045305169095,0.635);
#5643=TOROIDAL_SURFACE('',#100051,61.8704694830905,0.635);
#5644=TOROIDAL_SURFACE('',#100054,61.0131030316259,0.254);
#5645=TOROIDAL_SURFACE('',#100057,60.8618969683742,0.254);
#5646=TOROIDAL_SURFACE('',#100077,60.0045305169095,0.635);
#5647=TOROIDAL_SURFACE('',#100080,61.8704694830905,0.635);
#5648=TOROIDAL_SURFACE('',#100083,61.0131030316259,0.254);
#5649=TOROIDAL_SURFACE('',#100086,60.8618969683742,0.254);
#5650=TOROIDAL_SURFACE('',#100106,60.0045305169095,0.635);
#5651=TOROIDAL_SURFACE('',#100109,61.8704694830905,0.635);
#5652=TOROIDAL_SURFACE('',#100112,61.0131030316259,0.254);
#5653=TOROIDAL_SURFACE('',#100115,60.8618969683742,0.254);
#5654=TOROIDAL_SURFACE('',#100135,60.0045305169095,0.635);
#5655=TOROIDAL_SURFACE('',#100138,61.8704694830905,0.635);
#5656=TOROIDAL_SURFACE('',#100141,61.0131030316259,0.254);
#5657=TOROIDAL_SURFACE('',#100144,60.8618969683742,0.254);
#5658=TOROIDAL_SURFACE('',#100164,60.0045305169095,0.635);
#5659=TOROIDAL_SURFACE('',#100167,61.8704694830905,0.635);
#5660=TOROIDAL_SURFACE('',#100170,61.0131030316259,0.254);
#5661=TOROIDAL_SURFACE('',#100173,60.8618969683742,0.254);
#5662=TOROIDAL_SURFACE('',#100193,60.0045305169095,0.635);
#5663=TOROIDAL_SURFACE('',#100196,61.8704694830905,0.635);
#5664=TOROIDAL_SURFACE('',#100199,61.0131030316259,0.254);
#5665=TOROIDAL_SURFACE('',#100202,60.8618969683742,0.254);
#5666=TOROIDAL_SURFACE('',#100222,60.0045305169095,0.635);
#5667=TOROIDAL_SURFACE('',#100225,61.8704694830905,0.635);
#5668=TOROIDAL_SURFACE('',#100228,61.0131030316259,0.254);
#5669=TOROIDAL_SURFACE('',#100231,60.8618969683742,0.254);
#5670=TOROIDAL_SURFACE('',#100251,60.0045305169095,0.635);
#5671=TOROIDAL_SURFACE('',#100254,61.8704694830905,0.635);
#5672=TOROIDAL_SURFACE('',#100257,61.0131030316259,0.254);
#5673=TOROIDAL_SURFACE('',#100260,60.8618969683742,0.254);
#5674=TOROIDAL_SURFACE('',#100280,60.0045305169095,0.635);
#5675=TOROIDAL_SURFACE('',#100283,61.8704694830905,0.635);
#5676=TOROIDAL_SURFACE('',#100286,61.0131030316259,0.254);
#5677=TOROIDAL_SURFACE('',#100289,60.8618969683742,0.254);
#5678=TOROIDAL_SURFACE('',#100309,60.0045305169095,0.635);
#5679=TOROIDAL_SURFACE('',#100312,61.8704694830905,0.635);
#5680=TOROIDAL_SURFACE('',#100315,61.0131030316259,0.254);
#5681=TOROIDAL_SURFACE('',#100318,60.8618969683742,0.254);
#5682=TOROIDAL_SURFACE('',#100338,60.0045305169095,0.635);
#5683=TOROIDAL_SURFACE('',#100341,61.8704694830905,0.635);
#5684=TOROIDAL_SURFACE('',#100344,61.0131030316259,0.254);
#5685=TOROIDAL_SURFACE('',#100347,60.8618969683742,0.254);
#5686=TOROIDAL_SURFACE('',#100367,60.0045305169095,0.635);
#5687=TOROIDAL_SURFACE('',#100370,61.8704694830905,0.635);
#5688=TOROIDAL_SURFACE('',#100373,61.0131030316259,0.254);
#5689=TOROIDAL_SURFACE('',#100376,60.8618969683742,0.254);
#5690=TOROIDAL_SURFACE('',#100396,60.0045305169095,0.635);
#5691=TOROIDAL_SURFACE('',#100399,61.8704694830905,0.635);
#5692=TOROIDAL_SURFACE('',#100402,61.0131030316259,0.254);
#5693=TOROIDAL_SURFACE('',#100405,60.8618969683742,0.254);
#5694=TOROIDAL_SURFACE('',#100425,60.0045305169095,0.635);
#5695=TOROIDAL_SURFACE('',#100428,61.8704694830905,0.635);
#5696=TOROIDAL_SURFACE('',#100431,61.0131030316259,0.254);
#5697=TOROIDAL_SURFACE('',#100434,60.8618969683742,0.254);
#5698=TOROIDAL_SURFACE('',#100454,60.0045305169095,0.635);
#5699=TOROIDAL_SURFACE('',#100457,61.8704694830905,0.635);
#5700=TOROIDAL_SURFACE('',#100460,61.0131030316259,0.254);
#5701=TOROIDAL_SURFACE('',#100463,60.8618969683742,0.254);
#5702=TOROIDAL_SURFACE('',#100483,60.0045305169095,0.635);
#5703=TOROIDAL_SURFACE('',#100486,61.8704694830905,0.635);
#5704=TOROIDAL_SURFACE('',#100489,61.0131030316259,0.254);
#5705=TOROIDAL_SURFACE('',#100492,60.8618969683742,0.254);
#5706=TOROIDAL_SURFACE('',#100512,60.0045305169095,0.635);
#5707=TOROIDAL_SURFACE('',#100515,61.8704694830905,0.635);
#5708=TOROIDAL_SURFACE('',#100518,61.0131030316259,0.254);
#5709=TOROIDAL_SURFACE('',#100521,60.8618969683742,0.254);
#5710=TOROIDAL_SURFACE('',#100541,60.0045305169095,0.635);
#5711=TOROIDAL_SURFACE('',#100544,61.8704694830905,0.635);
#5712=TOROIDAL_SURFACE('',#100547,61.0131030316259,0.254);
#5713=TOROIDAL_SURFACE('',#100550,60.8618969683742,0.254);
#5714=TOROIDAL_SURFACE('',#100570,60.0045305169095,0.635);
#5715=TOROIDAL_SURFACE('',#100573,61.8704694830905,0.635);
#5716=TOROIDAL_SURFACE('',#100576,61.0131030316259,0.254);
#5717=TOROIDAL_SURFACE('',#100579,60.8618969683742,0.254);
#5718=TOROIDAL_SURFACE('',#100599,60.0045305169095,0.635);
#5719=TOROIDAL_SURFACE('',#100602,61.8704694830905,0.635);
#5720=TOROIDAL_SURFACE('',#100605,61.0131030316259,0.254);
#5721=TOROIDAL_SURFACE('',#100608,60.8618969683742,0.254);
#5722=TOROIDAL_SURFACE('',#100628,60.0045305169095,0.635);
#5723=TOROIDAL_SURFACE('',#100631,61.8704694830905,0.635);
#5724=TOROIDAL_SURFACE('',#100634,61.0131030316259,0.254);
#5725=TOROIDAL_SURFACE('',#100637,60.8618969683742,0.254);
#5726=TOROIDAL_SURFACE('',#100657,60.0045305169095,0.635);
#5727=TOROIDAL_SURFACE('',#100660,61.8704694830905,0.635);
#5728=TOROIDAL_SURFACE('',#100663,61.0131030316259,0.254);
#5729=TOROIDAL_SURFACE('',#100666,60.8618969683742,0.254);
#5730=TOROIDAL_SURFACE('',#100686,60.0045305169095,0.635);
#5731=TOROIDAL_SURFACE('',#100689,61.8704694830905,0.635);
#5732=TOROIDAL_SURFACE('',#100692,61.0131030316259,0.254);
#5733=TOROIDAL_SURFACE('',#100695,60.8618969683742,0.254);
#5734=TOROIDAL_SURFACE('',#100715,60.0045305169095,0.635);
#5735=TOROIDAL_SURFACE('',#100718,61.8704694830905,0.635);
#5736=TOROIDAL_SURFACE('',#100721,61.0131030316259,0.254);
#5737=TOROIDAL_SURFACE('',#100724,60.8618969683742,0.254);
#5738=TOROIDAL_SURFACE('',#100744,60.0045305169095,0.635);
#5739=TOROIDAL_SURFACE('',#100747,61.8704694830905,0.635);
#5740=TOROIDAL_SURFACE('',#100750,61.0131030316259,0.254);
#5741=TOROIDAL_SURFACE('',#100753,60.8618969683742,0.254);
#5742=TOROIDAL_SURFACE('',#100773,60.0045305169095,0.635);
#5743=TOROIDAL_SURFACE('',#100776,61.8704694830905,0.635);
#5744=TOROIDAL_SURFACE('',#100779,61.0131030316259,0.254);
#5745=TOROIDAL_SURFACE('',#100782,60.8618969683742,0.254);
#5746=TOROIDAL_SURFACE('',#100802,60.0045305169095,0.635);
#5747=TOROIDAL_SURFACE('',#100805,61.8704694830905,0.635);
#5748=TOROIDAL_SURFACE('',#100808,61.0131030316259,0.254);
#5749=TOROIDAL_SURFACE('',#100811,60.8618969683742,0.254);
#5750=TOROIDAL_SURFACE('',#100831,60.0045305169095,0.635);
#5751=TOROIDAL_SURFACE('',#100834,61.8704694830905,0.635);
#5752=TOROIDAL_SURFACE('',#100837,61.0131030316259,0.254);
#5753=TOROIDAL_SURFACE('',#100840,60.8618969683742,0.254);
#5754=TOROIDAL_SURFACE('',#100860,60.0045305169095,0.635);
#5755=TOROIDAL_SURFACE('',#100863,61.8704694830905,0.635);
#5756=TOROIDAL_SURFACE('',#100866,61.0131030316259,0.254);
#5757=TOROIDAL_SURFACE('',#100869,60.8618969683742,0.254);
#5758=TOROIDAL_SURFACE('',#100889,60.0045305169095,0.635);
#5759=TOROIDAL_SURFACE('',#100892,61.8704694830905,0.635);
#5760=TOROIDAL_SURFACE('',#100895,61.0131030316259,0.254);
#5761=TOROIDAL_SURFACE('',#100898,60.8618969683742,0.254);
#5762=TOROIDAL_SURFACE('',#100918,60.0045305169095,0.635);
#5763=TOROIDAL_SURFACE('',#100921,61.8704694830905,0.635);
#5764=TOROIDAL_SURFACE('',#100924,61.0131030316259,0.254);
#5765=TOROIDAL_SURFACE('',#100927,60.8618969683742,0.254);
#5766=TOROIDAL_SURFACE('',#100947,60.0045305169095,0.635);
#5767=TOROIDAL_SURFACE('',#100950,61.8704694830905,0.635);
#5768=TOROIDAL_SURFACE('',#100953,61.0131030316259,0.254);
#5769=TOROIDAL_SURFACE('',#100956,60.8618969683742,0.254);
#5770=TOROIDAL_SURFACE('',#100976,60.0045305169095,0.635);
#5771=TOROIDAL_SURFACE('',#100979,61.8704694830905,0.635);
#5772=TOROIDAL_SURFACE('',#100982,61.0131030316259,0.254);
#5773=TOROIDAL_SURFACE('',#100985,60.8618969683742,0.254);
#5774=TOROIDAL_SURFACE('',#101005,60.0045305169095,0.635);
#5775=TOROIDAL_SURFACE('',#101008,61.8704694830905,0.635);
#5776=TOROIDAL_SURFACE('',#101011,61.0131030316259,0.254);
#5777=TOROIDAL_SURFACE('',#101014,60.8618969683742,0.254);
#5778=TOROIDAL_SURFACE('',#101034,60.0045305169095,0.635);
#5779=TOROIDAL_SURFACE('',#101037,61.8704694830905,0.635);
#5780=TOROIDAL_SURFACE('',#101040,61.0131030316259,0.254);
#5781=TOROIDAL_SURFACE('',#101043,60.8618969683742,0.254);
#5782=TOROIDAL_SURFACE('',#101063,60.0045305169095,0.635);
#5783=TOROIDAL_SURFACE('',#101066,61.8704694830905,0.635);
#5784=TOROIDAL_SURFACE('',#101069,61.0131030316259,0.254);
#5785=TOROIDAL_SURFACE('',#101072,60.8618969683742,0.254);
#5786=TOROIDAL_SURFACE('',#101095,60.0045305169095,0.635);
#5787=TOROIDAL_SURFACE('',#101098,61.8704694830905,0.635);
#5788=TOROIDAL_SURFACE('',#101101,61.0131030316259,0.254);
#5789=TOROIDAL_SURFACE('',#101104,60.8618969683742,0.254);
#5790=TOROIDAL_SURFACE('',#101139,62.8464445485378,0.127);
#5791=TOROIDAL_SURFACE('',#101149,59.0285554514622,0.127);
#5792=TOROIDAL_SURFACE('',#102064,62.8464445485378,0.127);
#5793=TOROIDAL_SURFACE('',#102074,59.0285554514622,0.127);
#5794=TOROIDAL_SURFACE('',#102108,62.8464445485378,0.127);
#5795=TOROIDAL_SURFACE('',#102118,59.0285554514622,0.127);
#5796=TOROIDAL_SURFACE('',#102152,62.8464445485378,0.127);
#5797=TOROIDAL_SURFACE('',#102162,59.0285554514622,0.127);
#5798=TOROIDAL_SURFACE('',#102196,62.8464445485378,0.127);
#5799=TOROIDAL_SURFACE('',#102206,59.0285554514622,0.127);
#5800=TOROIDAL_SURFACE('',#102240,62.8464445485378,0.127);
#5801=TOROIDAL_SURFACE('',#102250,59.0285554514622,0.127);
#5802=TOROIDAL_SURFACE('',#102284,62.8464445485378,0.127);
#5803=TOROIDAL_SURFACE('',#102294,59.0285554514622,0.127);
#5804=TOROIDAL_SURFACE('',#102328,62.8464445485378,0.127);
#5805=TOROIDAL_SURFACE('',#102338,59.0285554514622,0.127);
#5806=TOROIDAL_SURFACE('',#102372,62.8464445485378,0.127);
#5807=TOROIDAL_SURFACE('',#102382,59.0285554514622,0.127);
#5808=TOROIDAL_SURFACE('',#102416,62.8464445485378,0.127);
#5809=TOROIDAL_SURFACE('',#102426,59.0285554514622,0.127);
#5810=TOROIDAL_SURFACE('',#102460,62.8464445485378,0.127);
#5811=TOROIDAL_SURFACE('',#102470,59.0285554514622,0.127);
#5812=TOROIDAL_SURFACE('',#102504,62.8464445485378,0.127);
#5813=TOROIDAL_SURFACE('',#102514,59.0285554514622,0.127);
#5814=TOROIDAL_SURFACE('',#102548,62.8464445485378,0.127);
#5815=TOROIDAL_SURFACE('',#102558,59.0285554514622,0.127);
#5816=TOROIDAL_SURFACE('',#102592,62.8464445485378,0.127);
#5817=TOROIDAL_SURFACE('',#102602,59.0285554514622,0.127);
#5818=TOROIDAL_SURFACE('',#102636,62.8464445485378,0.127);
#5819=TOROIDAL_SURFACE('',#102646,59.0285554514622,0.127);
#5820=TOROIDAL_SURFACE('',#102680,62.8464445485378,0.127);
#5821=TOROIDAL_SURFACE('',#102690,59.0285554514622,0.127);
#5822=TOROIDAL_SURFACE('',#102724,62.8464445485378,0.127);
#5823=TOROIDAL_SURFACE('',#102734,59.0285554514622,0.127);
#5824=TOROIDAL_SURFACE('',#102768,62.8464445485378,0.127);
#5825=TOROIDAL_SURFACE('',#102778,59.0285554514622,0.127);
#5826=TOROIDAL_SURFACE('',#102812,62.8464445485378,0.127);
#5827=TOROIDAL_SURFACE('',#102822,59.0285554514622,0.127);
#5828=TOROIDAL_SURFACE('',#102856,62.8464445485378,0.127);
#5829=TOROIDAL_SURFACE('',#102866,59.0285554514622,0.127);
#5830=TOROIDAL_SURFACE('',#102900,62.8464445485378,0.127);
#5831=TOROIDAL_SURFACE('',#102910,59.0285554514622,0.127);
#5832=TOROIDAL_SURFACE('',#102944,62.8464445485378,0.127);
#5833=TOROIDAL_SURFACE('',#102954,59.0285554514622,0.127);
#5834=TOROIDAL_SURFACE('',#102988,62.8464445485378,0.127);
#5835=TOROIDAL_SURFACE('',#102998,59.0285554514622,0.127);
#5836=TOROIDAL_SURFACE('',#103032,62.8464445485378,0.127);
#5837=TOROIDAL_SURFACE('',#103042,59.0285554514622,0.127);
#5838=TOROIDAL_SURFACE('',#103076,62.8464445485378,0.127);
#5839=TOROIDAL_SURFACE('',#103086,59.0285554514622,0.127);
#5840=TOROIDAL_SURFACE('',#103120,62.8464445485378,0.127);
#5841=TOROIDAL_SURFACE('',#103130,59.0285554514622,0.127);
#5842=TOROIDAL_SURFACE('',#103164,62.8464445485378,0.127);
#5843=TOROIDAL_SURFACE('',#103174,59.0285554514622,0.127);
#5844=TOROIDAL_SURFACE('',#103208,62.8464445485378,0.127);
#5845=TOROIDAL_SURFACE('',#103218,59.0285554514622,0.127);
#5846=TOROIDAL_SURFACE('',#103252,62.8464445485378,0.127);
#5847=TOROIDAL_SURFACE('',#103262,59.0285554514622,0.127);
#5848=TOROIDAL_SURFACE('',#103296,62.8464445485378,0.127);
#5849=TOROIDAL_SURFACE('',#103306,59.0285554514622,0.127);
#5850=TOROIDAL_SURFACE('',#103378,62.8464445485378,0.127);
#5851=TOROIDAL_SURFACE('',#103388,59.0285554514622,0.127);
#5852=TOROIDAL_SURFACE('',#103422,62.8464445485378,0.127);
#5853=TOROIDAL_SURFACE('',#103432,59.0285554514622,0.127);
#5854=TOROIDAL_SURFACE('',#103466,62.8464445485378,0.127);
#5855=TOROIDAL_SURFACE('',#103476,59.0285554514622,0.127);
#5856=TOROIDAL_SURFACE('',#103510,62.8464445485378,0.127);
#5857=TOROIDAL_SURFACE('',#103520,59.0285554514622,0.127);
#5858=TOROIDAL_SURFACE('',#103554,62.8464445485378,0.127);
#5859=TOROIDAL_SURFACE('',#103564,59.0285554514622,0.127);
#5860=TOROIDAL_SURFACE('',#103598,62.8464445485378,0.127);
#5861=TOROIDAL_SURFACE('',#103608,59.0285554514622,0.127);
#5862=TOROIDAL_SURFACE('',#103642,62.8464445485378,0.127);
#5863=TOROIDAL_SURFACE('',#103652,59.0285554514622,0.127);
#5864=TOROIDAL_SURFACE('',#103686,62.8464445485378,0.127);
#5865=TOROIDAL_SURFACE('',#103696,59.0285554514622,0.127);
#5866=TOROIDAL_SURFACE('',#103730,62.8464445485378,0.127);
#5867=TOROIDAL_SURFACE('',#103740,59.0285554514622,0.127);
#5868=TOROIDAL_SURFACE('',#103774,62.8464445485378,0.127);
#5869=TOROIDAL_SURFACE('',#103784,59.0285554514622,0.127);
#5870=TOROIDAL_SURFACE('',#103818,62.8464445485378,0.127);
#5871=TOROIDAL_SURFACE('',#103828,59.0285554514622,0.127);
#5872=TOROIDAL_SURFACE('',#103862,62.8464445485378,0.127);
#5873=TOROIDAL_SURFACE('',#103872,59.0285554514622,0.127);
#5874=TOROIDAL_SURFACE('',#103906,62.8464445485378,0.127);
#5875=TOROIDAL_SURFACE('',#103916,59.0285554514622,0.127);
#5876=TOROIDAL_SURFACE('',#103950,62.8464445485378,0.127);
#5877=TOROIDAL_SURFACE('',#103960,59.0285554514622,0.127);
#5878=TOROIDAL_SURFACE('',#104032,62.8464445485378,0.127);
#5879=TOROIDAL_SURFACE('',#104042,59.0285554514622,0.127);
#5880=TOROIDAL_SURFACE('',#104076,62.8464445485378,0.127);
#5881=TOROIDAL_SURFACE('',#104086,59.0285554514622,0.127);
#5882=TOROIDAL_SURFACE('',#104120,62.8464445485378,0.127);
#5883=TOROIDAL_SURFACE('',#104130,59.0285554514622,0.127);
#5884=TOROIDAL_SURFACE('',#104164,62.8464445485378,0.127);
#5885=TOROIDAL_SURFACE('',#104174,59.0285554514622,0.127);
#5886=TOROIDAL_SURFACE('',#104208,62.8464445485378,0.127);
#5887=TOROIDAL_SURFACE('',#104218,59.0285554514622,0.127);
#5888=TOROIDAL_SURFACE('',#104252,62.8464445485378,0.127);
#5889=TOROIDAL_SURFACE('',#104262,59.0285554514622,0.127);
#5890=TOROIDAL_SURFACE('',#104296,62.8464445485378,0.127);
#5891=TOROIDAL_SURFACE('',#104306,59.0285554514622,0.127);
#5892=TOROIDAL_SURFACE('',#104340,62.8464445485378,0.127);
#5893=TOROIDAL_SURFACE('',#104350,59.0285554514622,0.127);
#5894=TOROIDAL_SURFACE('',#104384,62.8464445485378,0.127);
#5895=TOROIDAL_SURFACE('',#104394,59.0285554514622,0.127);
#5896=TOROIDAL_SURFACE('',#104428,62.8464445485378,0.127);
#5897=TOROIDAL_SURFACE('',#104438,59.0285554514622,0.127);
#5898=TOROIDAL_SURFACE('',#104472,62.8464445485378,0.127);
#5899=TOROIDAL_SURFACE('',#104482,59.0285554514622,0.127);
#5900=TOROIDAL_SURFACE('',#104516,62.8464445485378,0.127);
#5901=TOROIDAL_SURFACE('',#104526,59.0285554514622,0.127);
#5902=TOROIDAL_SURFACE('',#104560,62.8464445485378,0.127);
#5903=TOROIDAL_SURFACE('',#104570,59.0285554514622,0.127);
#5904=TOROIDAL_SURFACE('',#104604,62.8464445485378,0.127);
#5905=TOROIDAL_SURFACE('',#104614,59.0285554514622,0.127);
#5906=TOROIDAL_SURFACE('',#104631,59.0285554514622,0.127);
#5907=TOROIDAL_SURFACE('',#104636,62.8464445485378,0.127);
#5908=TOROIDAL_SURFACE('',#104641,59.0285554514622,0.127);
#5909=TOROIDAL_SURFACE('',#104646,62.8464445485378,0.127);
#5910=TOROIDAL_SURFACE('',#104652,58.2189663438286,0.635);
#5911=TOROIDAL_SURFACE('',#104657,58.3085779254084,0.635);
#5912=TOROIDAL_SURFACE('',#104661,63.5664220745916,0.635);
#5913=TOROIDAL_SURFACE('',#104666,63.6560336561714,0.635);
#5914=TOROIDAL_SURFACE('',#104935,60.0045305169095,0.635);
#5915=TOROIDAL_SURFACE('',#104938,61.8704694830905,0.635);
#5916=TOROIDAL_SURFACE('',#104941,61.0131030316259,0.254);
#5917=TOROIDAL_SURFACE('',#104944,60.8618969683742,0.254);
#5918=TOROIDAL_SURFACE('',#104964,60.0045305169095,0.635);
#5919=TOROIDAL_SURFACE('',#104967,61.8704694830905,0.635);
#5920=TOROIDAL_SURFACE('',#104970,61.0131030316259,0.254);
#5921=TOROIDAL_SURFACE('',#104973,60.8618969683742,0.254);
#5922=TOROIDAL_SURFACE('',#104993,60.0045305169095,0.635);
#5923=TOROIDAL_SURFACE('',#104996,61.8704694830905,0.635);
#5924=TOROIDAL_SURFACE('',#104999,61.0131030316259,0.254);
#5925=TOROIDAL_SURFACE('',#105002,60.8618969683742,0.254);
#5926=TOROIDAL_SURFACE('',#105022,60.0045305169095,0.635);
#5927=TOROIDAL_SURFACE('',#105025,61.8704694830905,0.635);
#5928=TOROIDAL_SURFACE('',#105028,61.0131030316259,0.254);
#5929=TOROIDAL_SURFACE('',#105031,60.8618969683742,0.254);
#5930=TOROIDAL_SURFACE('',#105051,60.0045305169095,0.635);
#5931=TOROIDAL_SURFACE('',#105054,61.8704694830905,0.635);
#5932=TOROIDAL_SURFACE('',#105057,61.0131030316259,0.254);
#5933=TOROIDAL_SURFACE('',#105060,60.8618969683742,0.254);
#5934=TOROIDAL_SURFACE('',#105080,60.0045305169095,0.635);
#5935=TOROIDAL_SURFACE('',#105083,61.8704694830905,0.635);
#5936=TOROIDAL_SURFACE('',#105086,61.0131030316259,0.254);
#5937=TOROIDAL_SURFACE('',#105089,60.8618969683742,0.254);
#5938=TOROIDAL_SURFACE('',#105109,60.0045305169095,0.635);
#5939=TOROIDAL_SURFACE('',#105112,61.8704694830905,0.635);
#5940=TOROIDAL_SURFACE('',#105115,61.0131030316259,0.254);
#5941=TOROIDAL_SURFACE('',#105118,60.8618969683742,0.254);
#5942=TOROIDAL_SURFACE('',#105138,60.0045305169095,0.635);
#5943=TOROIDAL_SURFACE('',#105141,61.8704694830905,0.635);
#5944=TOROIDAL_SURFACE('',#105144,61.0131030316259,0.254);
#5945=TOROIDAL_SURFACE('',#105147,60.8618969683742,0.254);
#5946=TOROIDAL_SURFACE('',#105167,60.0045305169095,0.635);
#5947=TOROIDAL_SURFACE('',#105170,61.8704694830905,0.635);
#5948=TOROIDAL_SURFACE('',#105173,61.0131030316259,0.254);
#5949=TOROIDAL_SURFACE('',#105176,60.8618969683742,0.254);
#5950=TOROIDAL_SURFACE('',#105196,60.0045305169095,0.635);
#5951=TOROIDAL_SURFACE('',#105199,61.8704694830905,0.635);
#5952=TOROIDAL_SURFACE('',#105202,61.0131030316259,0.254);
#5953=TOROIDAL_SURFACE('',#105205,60.8618969683742,0.254);
#5954=TOROIDAL_SURFACE('',#105225,60.0045305169095,0.635);
#5955=TOROIDAL_SURFACE('',#105228,61.8704694830905,0.635);
#5956=TOROIDAL_SURFACE('',#105231,61.0131030316259,0.254);
#5957=TOROIDAL_SURFACE('',#105234,60.8618969683742,0.254);
#5958=TOROIDAL_SURFACE('',#105254,60.0045305169095,0.635);
#5959=TOROIDAL_SURFACE('',#105257,61.8704694830905,0.635);
#5960=TOROIDAL_SURFACE('',#105260,61.0131030316259,0.254);
#5961=TOROIDAL_SURFACE('',#105263,60.8618969683742,0.254);
#5962=TOROIDAL_SURFACE('',#105283,60.0045305169095,0.635);
#5963=TOROIDAL_SURFACE('',#105286,61.8704694830905,0.635);
#5964=TOROIDAL_SURFACE('',#105289,61.0131030316259,0.254);
#5965=TOROIDAL_SURFACE('',#105292,60.8618969683742,0.254);
#5966=TOROIDAL_SURFACE('',#105312,60.0045305169095,0.635);
#5967=TOROIDAL_SURFACE('',#105315,61.8704694830905,0.635);
#5968=TOROIDAL_SURFACE('',#105318,61.0131030316259,0.254);
#5969=TOROIDAL_SURFACE('',#105321,60.8618969683742,0.254);
#5970=TOROIDAL_SURFACE('',#105341,60.0045305169095,0.635);
#5971=TOROIDAL_SURFACE('',#105344,61.8704694830905,0.635);
#5972=TOROIDAL_SURFACE('',#105347,61.0131030316259,0.254);
#5973=TOROIDAL_SURFACE('',#105350,60.8618969683742,0.254);
#5974=TOROIDAL_SURFACE('',#105370,60.0045305169095,0.635);
#5975=TOROIDAL_SURFACE('',#105373,61.8704694830905,0.635);
#5976=TOROIDAL_SURFACE('',#105376,61.0131030316259,0.254);
#5977=TOROIDAL_SURFACE('',#105379,60.8618969683742,0.254);
#5978=TOROIDAL_SURFACE('',#105399,60.0045305169095,0.635);
#5979=TOROIDAL_SURFACE('',#105402,61.8704694830905,0.635);
#5980=TOROIDAL_SURFACE('',#105405,61.0131030316259,0.254);
#5981=TOROIDAL_SURFACE('',#105408,60.8618969683742,0.254);
#5982=TOROIDAL_SURFACE('',#105428,60.0045305169095,0.635);
#5983=TOROIDAL_SURFACE('',#105431,61.8704694830905,0.635);
#5984=TOROIDAL_SURFACE('',#105434,61.0131030316259,0.254);
#5985=TOROIDAL_SURFACE('',#105437,60.8618969683742,0.254);
#5986=TOROIDAL_SURFACE('',#105457,60.0045305169095,0.635);
#5987=TOROIDAL_SURFACE('',#105460,61.8704694830905,0.635);
#5988=TOROIDAL_SURFACE('',#105463,61.0131030316259,0.254);
#5989=TOROIDAL_SURFACE('',#105466,60.8618969683742,0.254);
#5990=TOROIDAL_SURFACE('',#105486,60.0045305169095,0.635);
#5991=TOROIDAL_SURFACE('',#105489,61.8704694830905,0.635);
#5992=TOROIDAL_SURFACE('',#105492,61.0131030316259,0.254);
#5993=TOROIDAL_SURFACE('',#105495,60.8618969683742,0.254);
#5994=TOROIDAL_SURFACE('',#105515,60.0045305169095,0.635);
#5995=TOROIDAL_SURFACE('',#105518,61.8704694830905,0.635);
#5996=TOROIDAL_SURFACE('',#105521,61.0131030316259,0.254);
#5997=TOROIDAL_SURFACE('',#105524,60.8618969683742,0.254);
#5998=TOROIDAL_SURFACE('',#105544,60.0045305169095,0.635);
#5999=TOROIDAL_SURFACE('',#105547,61.8704694830905,0.635);
#6000=TOROIDAL_SURFACE('',#105550,61.0131030316259,0.254);
#6001=TOROIDAL_SURFACE('',#105553,60.8618969683742,0.254);
#6002=TOROIDAL_SURFACE('',#105573,60.0045305169095,0.635);
#6003=TOROIDAL_SURFACE('',#105576,61.8704694830905,0.635);
#6004=TOROIDAL_SURFACE('',#105579,61.0131030316259,0.254);
#6005=TOROIDAL_SURFACE('',#105582,60.8618969683742,0.254);
#6006=TOROIDAL_SURFACE('',#105602,60.0045305169095,0.635);
#6007=TOROIDAL_SURFACE('',#105605,61.8704694830905,0.635);
#6008=TOROIDAL_SURFACE('',#105608,61.0131030316259,0.254);
#6009=TOROIDAL_SURFACE('',#105611,60.8618969683742,0.254);
#6010=TOROIDAL_SURFACE('',#105631,60.0045305169095,0.635);
#6011=TOROIDAL_SURFACE('',#105634,61.8704694830905,0.635);
#6012=TOROIDAL_SURFACE('',#105637,61.0131030316259,0.254);
#6013=TOROIDAL_SURFACE('',#105640,60.8618969683742,0.254);
#6014=TOROIDAL_SURFACE('',#105660,60.0045305169095,0.635);
#6015=TOROIDAL_SURFACE('',#105663,61.8704694830905,0.635);
#6016=TOROIDAL_SURFACE('',#105666,61.0131030316259,0.254);
#6017=TOROIDAL_SURFACE('',#105669,60.8618969683742,0.254);
#6018=TOROIDAL_SURFACE('',#105689,60.0045305169095,0.635);
#6019=TOROIDAL_SURFACE('',#105692,61.8704694830905,0.635);
#6020=TOROIDAL_SURFACE('',#105695,61.0131030316259,0.254);
#6021=TOROIDAL_SURFACE('',#105698,60.8618969683742,0.254);
#6022=TOROIDAL_SURFACE('',#105718,60.0045305169095,0.635);
#6023=TOROIDAL_SURFACE('',#105721,61.8704694830905,0.635);
#6024=TOROIDAL_SURFACE('',#105724,61.0131030316259,0.254);
#6025=TOROIDAL_SURFACE('',#105727,60.8618969683742,0.254);
#6026=TOROIDAL_SURFACE('',#105747,60.0045305169095,0.635);
#6027=TOROIDAL_SURFACE('',#105750,61.8704694830905,0.635);
#6028=TOROIDAL_SURFACE('',#105753,61.0131030316259,0.254);
#6029=TOROIDAL_SURFACE('',#105756,60.8618969683742,0.254);
#6030=TOROIDAL_SURFACE('',#105776,60.0045305169095,0.635);
#6031=TOROIDAL_SURFACE('',#105779,61.8704694830905,0.635);
#6032=TOROIDAL_SURFACE('',#105782,61.0131030316259,0.254);
#6033=TOROIDAL_SURFACE('',#105785,60.8618969683742,0.254);
#6034=TOROIDAL_SURFACE('',#105805,60.0045305169095,0.635);
#6035=TOROIDAL_SURFACE('',#105808,61.8704694830905,0.635);
#6036=TOROIDAL_SURFACE('',#105811,61.0131030316259,0.254);
#6037=TOROIDAL_SURFACE('',#105814,60.8618969683742,0.254);
#6038=TOROIDAL_SURFACE('',#105834,60.0045305169095,0.635);
#6039=TOROIDAL_SURFACE('',#105837,61.8704694830905,0.635);
#6040=TOROIDAL_SURFACE('',#105840,61.0131030316259,0.254);
#6041=TOROIDAL_SURFACE('',#105843,60.8618969683742,0.254);
#6042=TOROIDAL_SURFACE('',#105863,60.0045305169095,0.635);
#6043=TOROIDAL_SURFACE('',#105866,61.8704694830905,0.635);
#6044=TOROIDAL_SURFACE('',#105869,61.0131030316259,0.254);
#6045=TOROIDAL_SURFACE('',#105872,60.8618969683742,0.254);
#6046=TOROIDAL_SURFACE('',#105892,60.0045305169095,0.635);
#6047=TOROIDAL_SURFACE('',#105895,61.8704694830905,0.635);
#6048=TOROIDAL_SURFACE('',#105898,61.0131030316259,0.254);
#6049=TOROIDAL_SURFACE('',#105901,60.8618969683742,0.254);
#6050=TOROIDAL_SURFACE('',#105921,60.0045305169095,0.635);
#6051=TOROIDAL_SURFACE('',#105924,61.8704694830905,0.635);
#6052=TOROIDAL_SURFACE('',#105927,61.0131030316259,0.254);
#6053=TOROIDAL_SURFACE('',#105930,60.8618969683742,0.254);
#6054=TOROIDAL_SURFACE('',#105950,60.0045305169095,0.635);
#6055=TOROIDAL_SURFACE('',#105953,61.8704694830905,0.635);
#6056=TOROIDAL_SURFACE('',#105956,61.0131030316259,0.254);
#6057=TOROIDAL_SURFACE('',#105959,60.8618969683742,0.254);
#6058=TOROIDAL_SURFACE('',#105979,60.0045305169095,0.635);
#6059=TOROIDAL_SURFACE('',#105982,61.8704694830905,0.635);
#6060=TOROIDAL_SURFACE('',#105985,61.0131030316259,0.254);
#6061=TOROIDAL_SURFACE('',#105988,60.8618969683742,0.254);
#6062=TOROIDAL_SURFACE('',#106008,60.0045305169095,0.635);
#6063=TOROIDAL_SURFACE('',#106011,61.8704694830905,0.635);
#6064=TOROIDAL_SURFACE('',#106014,61.0131030316259,0.254);
#6065=TOROIDAL_SURFACE('',#106017,60.8618969683742,0.254);
#6066=TOROIDAL_SURFACE('',#106037,60.0045305169095,0.635);
#6067=TOROIDAL_SURFACE('',#106040,61.8704694830905,0.635);
#6068=TOROIDAL_SURFACE('',#106043,61.0131030316259,0.254);
#6069=TOROIDAL_SURFACE('',#106046,60.8618969683742,0.254);
#6070=TOROIDAL_SURFACE('',#106066,60.0045305169095,0.635);
#6071=TOROIDAL_SURFACE('',#106069,61.8704694830905,0.635);
#6072=TOROIDAL_SURFACE('',#106072,61.0131030316259,0.254);
#6073=TOROIDAL_SURFACE('',#106075,60.8618969683742,0.254);
#6074=TOROIDAL_SURFACE('',#106095,60.0045305169095,0.635);
#6075=TOROIDAL_SURFACE('',#106098,61.8704694830905,0.635);
#6076=TOROIDAL_SURFACE('',#106101,61.0131030316259,0.254);
#6077=TOROIDAL_SURFACE('',#106104,60.8618969683742,0.254);
#6078=TOROIDAL_SURFACE('',#106124,60.0045305169095,0.635);
#6079=TOROIDAL_SURFACE('',#106127,61.8704694830905,0.635);
#6080=TOROIDAL_SURFACE('',#106130,61.0131030316259,0.254);
#6081=TOROIDAL_SURFACE('',#106133,60.8618969683742,0.254);
#6082=TOROIDAL_SURFACE('',#106153,60.0045305169095,0.635);
#6083=TOROIDAL_SURFACE('',#106156,61.8704694830905,0.635);
#6084=TOROIDAL_SURFACE('',#106159,61.0131030316259,0.254);
#6085=TOROIDAL_SURFACE('',#106162,60.8618969683742,0.254);
#6086=TOROIDAL_SURFACE('',#106182,60.0045305169095,0.635);
#6087=TOROIDAL_SURFACE('',#106185,61.8704694830905,0.635);
#6088=TOROIDAL_SURFACE('',#106188,61.0131030316259,0.254);
#6089=TOROIDAL_SURFACE('',#106191,60.8618969683742,0.254);
#6090=TOROIDAL_SURFACE('',#106211,60.0045305169095,0.635);
#6091=TOROIDAL_SURFACE('',#106214,61.8704694830905,0.635);
#6092=TOROIDAL_SURFACE('',#106217,61.0131030316259,0.254);
#6093=TOROIDAL_SURFACE('',#106220,60.8618969683742,0.254);
#6094=TOROIDAL_SURFACE('',#106240,60.0045305169095,0.635);
#6095=TOROIDAL_SURFACE('',#106243,61.8704694830905,0.635);
#6096=TOROIDAL_SURFACE('',#106246,61.0131030316259,0.254);
#6097=TOROIDAL_SURFACE('',#106249,60.8618969683742,0.254);
#6098=TOROIDAL_SURFACE('',#106269,60.0045305169095,0.635);
#6099=TOROIDAL_SURFACE('',#106272,61.8704694830905,0.635);
#6100=TOROIDAL_SURFACE('',#106275,61.0131030316259,0.254);
#6101=TOROIDAL_SURFACE('',#106278,60.8618969683742,0.254);
#6102=TOROIDAL_SURFACE('',#106298,60.0045305169095,0.635);
#6103=TOROIDAL_SURFACE('',#106301,61.8704694830905,0.635);
#6104=TOROIDAL_SURFACE('',#106304,61.0131030316259,0.254);
#6105=TOROIDAL_SURFACE('',#106307,60.8618969683742,0.254);
#6106=TOROIDAL_SURFACE('',#106327,60.0045305169095,0.635);
#6107=TOROIDAL_SURFACE('',#106330,61.8704694830905,0.635);
#6108=TOROIDAL_SURFACE('',#106333,61.0131030316259,0.254);
#6109=TOROIDAL_SURFACE('',#106336,60.8618969683742,0.254);
#6110=TOROIDAL_SURFACE('',#106356,60.0045305169095,0.635);
#6111=TOROIDAL_SURFACE('',#106359,61.8704694830905,0.635);
#6112=TOROIDAL_SURFACE('',#106362,61.0131030316259,0.254);
#6113=TOROIDAL_SURFACE('',#106365,60.8618969683742,0.254);
#6114=TOROIDAL_SURFACE('',#106385,60.0045305169095,0.635);
#6115=TOROIDAL_SURFACE('',#106388,61.8704694830905,0.635);
#6116=TOROIDAL_SURFACE('',#106391,61.0131030316259,0.254);
#6117=TOROIDAL_SURFACE('',#106394,60.8618969683742,0.254);
#6118=TOROIDAL_SURFACE('',#106414,60.0045305169095,0.635);
#6119=TOROIDAL_SURFACE('',#106417,61.8704694830905,0.635);
#6120=TOROIDAL_SURFACE('',#106420,61.0131030316259,0.254);
#6121=TOROIDAL_SURFACE('',#106423,60.8618969683742,0.254);
#6122=TOROIDAL_SURFACE('',#106443,60.0045305169095,0.635);
#6123=TOROIDAL_SURFACE('',#106446,61.8704694830905,0.635);
#6124=TOROIDAL_SURFACE('',#106449,61.0131030316259,0.254);
#6125=TOROIDAL_SURFACE('',#106452,60.8618969683742,0.254);
#6126=TOROIDAL_SURFACE('',#106472,60.0045305169095,0.635);
#6127=TOROIDAL_SURFACE('',#106475,61.8704694830905,0.635);
#6128=TOROIDAL_SURFACE('',#106478,61.0131030316259,0.254);
#6129=TOROIDAL_SURFACE('',#106481,60.8618969683742,0.254);
#6130=TOROIDAL_SURFACE('',#106501,60.0045305169095,0.635);
#6131=TOROIDAL_SURFACE('',#106504,61.8704694830905,0.635);
#6132=TOROIDAL_SURFACE('',#106507,61.0131030316259,0.254);
#6133=TOROIDAL_SURFACE('',#106510,60.8618969683742,0.254);
#6134=TOROIDAL_SURFACE('',#106530,60.0045305169095,0.635);
#6135=TOROIDAL_SURFACE('',#106533,61.8704694830905,0.635);
#6136=TOROIDAL_SURFACE('',#106536,61.0131030316259,0.254);
#6137=TOROIDAL_SURFACE('',#106539,60.8618969683742,0.254);
#6138=TOROIDAL_SURFACE('',#106559,60.0045305169095,0.635);
#6139=TOROIDAL_SURFACE('',#106562,61.8704694830905,0.635);
#6140=TOROIDAL_SURFACE('',#106565,61.0131030316259,0.254);
#6141=TOROIDAL_SURFACE('',#106568,60.8618969683742,0.254);
#6142=TOROIDAL_SURFACE('',#106588,60.0045305169095,0.635);
#6143=TOROIDAL_SURFACE('',#106591,61.8704694830905,0.635);
#6144=TOROIDAL_SURFACE('',#106594,61.0131030316259,0.254);
#6145=TOROIDAL_SURFACE('',#106597,60.8618969683742,0.254);
#6146=TOROIDAL_SURFACE('',#106617,60.0045305169095,0.635);
#6147=TOROIDAL_SURFACE('',#106620,61.8704694830905,0.635);
#6148=TOROIDAL_SURFACE('',#106623,61.0131030316259,0.254);
#6149=TOROIDAL_SURFACE('',#106626,60.8618969683742,0.254);
#6150=TOROIDAL_SURFACE('',#106649,60.0045305169095,0.635);
#6151=TOROIDAL_SURFACE('',#106652,61.8704694830905,0.635);
#6152=TOROIDAL_SURFACE('',#106655,61.0131030316259,0.254);
#6153=TOROIDAL_SURFACE('',#106658,60.8618969683742,0.254);
#6154=TOROIDAL_SURFACE('',#106693,62.8464445485378,0.127);
#6155=TOROIDAL_SURFACE('',#106703,59.0285554514622,0.127);
#6156=TOROIDAL_SURFACE('',#107618,62.8464445485378,0.127);
#6157=TOROIDAL_SURFACE('',#107628,59.0285554514622,0.127);
#6158=TOROIDAL_SURFACE('',#107662,62.8464445485378,0.127);
#6159=TOROIDAL_SURFACE('',#107672,59.0285554514622,0.127);
#6160=TOROIDAL_SURFACE('',#107706,62.8464445485378,0.127);
#6161=TOROIDAL_SURFACE('',#107716,59.0285554514622,0.127);
#6162=TOROIDAL_SURFACE('',#107750,62.8464445485378,0.127);
#6163=TOROIDAL_SURFACE('',#107760,59.0285554514622,0.127);
#6164=TOROIDAL_SURFACE('',#107794,62.8464445485378,0.127);
#6165=TOROIDAL_SURFACE('',#107804,59.0285554514622,0.127);
#6166=TOROIDAL_SURFACE('',#107838,62.8464445485378,0.127);
#6167=TOROIDAL_SURFACE('',#107848,59.0285554514622,0.127);
#6168=TOROIDAL_SURFACE('',#107882,62.8464445485378,0.127);
#6169=TOROIDAL_SURFACE('',#107892,59.0285554514622,0.127);
#6170=TOROIDAL_SURFACE('',#107926,62.8464445485378,0.127);
#6171=TOROIDAL_SURFACE('',#107936,59.0285554514622,0.127);
#6172=TOROIDAL_SURFACE('',#107970,62.8464445485378,0.127);
#6173=TOROIDAL_SURFACE('',#107980,59.0285554514622,0.127);
#6174=TOROIDAL_SURFACE('',#108014,62.8464445485378,0.127);
#6175=TOROIDAL_SURFACE('',#108024,59.0285554514622,0.127);
#6176=TOROIDAL_SURFACE('',#108058,62.8464445485378,0.127);
#6177=TOROIDAL_SURFACE('',#108068,59.0285554514622,0.127);
#6178=TOROIDAL_SURFACE('',#108102,62.8464445485378,0.127);
#6179=TOROIDAL_SURFACE('',#108112,59.0285554514622,0.127);
#6180=TOROIDAL_SURFACE('',#108146,62.8464445485378,0.127);
#6181=TOROIDAL_SURFACE('',#108156,59.0285554514622,0.127);
#6182=TOROIDAL_SURFACE('',#108190,62.8464445485378,0.127);
#6183=TOROIDAL_SURFACE('',#108200,59.0285554514622,0.127);
#6184=TOROIDAL_SURFACE('',#108234,62.8464445485378,0.127);
#6185=TOROIDAL_SURFACE('',#108244,59.0285554514622,0.127);
#6186=TOROIDAL_SURFACE('',#108278,62.8464445485378,0.127);
#6187=TOROIDAL_SURFACE('',#108288,59.0285554514622,0.127);
#6188=TOROIDAL_SURFACE('',#108322,62.8464445485378,0.127);
#6189=TOROIDAL_SURFACE('',#108332,59.0285554514622,0.127);
#6190=TOROIDAL_SURFACE('',#108366,62.8464445485378,0.127);
#6191=TOROIDAL_SURFACE('',#108376,59.0285554514622,0.127);
#6192=TOROIDAL_SURFACE('',#108410,62.8464445485378,0.127);
#6193=TOROIDAL_SURFACE('',#108420,59.0285554514622,0.127);
#6194=TOROIDAL_SURFACE('',#108454,62.8464445485378,0.127);
#6195=TOROIDAL_SURFACE('',#108464,59.0285554514622,0.127);
#6196=TOROIDAL_SURFACE('',#108498,62.8464445485378,0.127);
#6197=TOROIDAL_SURFACE('',#108508,59.0285554514622,0.127);
#6198=TOROIDAL_SURFACE('',#108542,62.8464445485378,0.127);
#6199=TOROIDAL_SURFACE('',#108552,59.0285554514622,0.127);
#6200=TOROIDAL_SURFACE('',#108586,62.8464445485378,0.127);
#6201=TOROIDAL_SURFACE('',#108596,59.0285554514622,0.127);
#6202=TOROIDAL_SURFACE('',#108630,62.8464445485378,0.127);
#6203=TOROIDAL_SURFACE('',#108640,59.0285554514622,0.127);
#6204=TOROIDAL_SURFACE('',#108674,62.8464445485378,0.127);
#6205=TOROIDAL_SURFACE('',#108684,59.0285554514622,0.127);
#6206=TOROIDAL_SURFACE('',#108718,62.8464445485378,0.127);
#6207=TOROIDAL_SURFACE('',#108728,59.0285554514622,0.127);
#6208=TOROIDAL_SURFACE('',#108762,62.8464445485378,0.127);
#6209=TOROIDAL_SURFACE('',#108772,59.0285554514622,0.127);
#6210=TOROIDAL_SURFACE('',#108806,62.8464445485378,0.127);
#6211=TOROIDAL_SURFACE('',#108816,59.0285554514622,0.127);
#6212=TOROIDAL_SURFACE('',#108850,62.8464445485378,0.127);
#6213=TOROIDAL_SURFACE('',#108860,59.0285554514622,0.127);
#6214=TOROIDAL_SURFACE('',#108932,62.8464445485378,0.127);
#6215=TOROIDAL_SURFACE('',#108942,59.0285554514622,0.127);
#6216=TOROIDAL_SURFACE('',#108976,62.8464445485378,0.127);
#6217=TOROIDAL_SURFACE('',#108986,59.0285554514622,0.127);
#6218=TOROIDAL_SURFACE('',#109020,62.8464445485378,0.127);
#6219=TOROIDAL_SURFACE('',#109030,59.0285554514622,0.127);
#6220=TOROIDAL_SURFACE('',#109064,62.8464445485378,0.127);
#6221=TOROIDAL_SURFACE('',#109074,59.0285554514622,0.127);
#6222=TOROIDAL_SURFACE('',#109108,62.8464445485378,0.127);
#6223=TOROIDAL_SURFACE('',#109118,59.0285554514622,0.127);
#6224=TOROIDAL_SURFACE('',#109152,62.8464445485378,0.127);
#6225=TOROIDAL_SURFACE('',#109162,59.0285554514622,0.127);
#6226=TOROIDAL_SURFACE('',#109196,62.8464445485378,0.127);
#6227=TOROIDAL_SURFACE('',#109206,59.0285554514622,0.127);
#6228=TOROIDAL_SURFACE('',#109240,62.8464445485378,0.127);
#6229=TOROIDAL_SURFACE('',#109250,59.0285554514622,0.127);
#6230=TOROIDAL_SURFACE('',#109284,62.8464445485378,0.127);
#6231=TOROIDAL_SURFACE('',#109294,59.0285554514622,0.127);
#6232=TOROIDAL_SURFACE('',#109328,62.8464445485378,0.127);
#6233=TOROIDAL_SURFACE('',#109338,59.0285554514622,0.127);
#6234=TOROIDAL_SURFACE('',#109372,62.8464445485378,0.127);
#6235=TOROIDAL_SURFACE('',#109382,59.0285554514622,0.127);
#6236=TOROIDAL_SURFACE('',#109416,62.8464445485378,0.127);
#6237=TOROIDAL_SURFACE('',#109426,59.0285554514622,0.127);
#6238=TOROIDAL_SURFACE('',#109460,62.8464445485378,0.127);
#6239=TOROIDAL_SURFACE('',#109470,59.0285554514622,0.127);
#6240=TOROIDAL_SURFACE('',#109504,62.8464445485378,0.127);
#6241=TOROIDAL_SURFACE('',#109514,59.0285554514622,0.127);
#6242=TOROIDAL_SURFACE('',#109586,62.8464445485378,0.127);
#6243=TOROIDAL_SURFACE('',#109596,59.0285554514622,0.127);
#6244=TOROIDAL_SURFACE('',#109630,62.8464445485378,0.127);
#6245=TOROIDAL_SURFACE('',#109640,59.0285554514622,0.127);
#6246=TOROIDAL_SURFACE('',#109674,62.8464445485378,0.127);
#6247=TOROIDAL_SURFACE('',#109684,59.0285554514622,0.127);
#6248=TOROIDAL_SURFACE('',#109718,62.8464445485378,0.127);
#6249=TOROIDAL_SURFACE('',#109728,59.0285554514622,0.127);
#6250=TOROIDAL_SURFACE('',#109762,62.8464445485378,0.127);
#6251=TOROIDAL_SURFACE('',#109772,59.0285554514622,0.127);
#6252=TOROIDAL_SURFACE('',#109806,62.8464445485378,0.127);
#6253=TOROIDAL_SURFACE('',#109816,59.0285554514622,0.127);
#6254=TOROIDAL_SURFACE('',#109850,62.8464445485378,0.127);
#6255=TOROIDAL_SURFACE('',#109860,59.0285554514622,0.127);
#6256=TOROIDAL_SURFACE('',#109894,62.8464445485378,0.127);
#6257=TOROIDAL_SURFACE('',#109904,59.0285554514622,0.127);
#6258=TOROIDAL_SURFACE('',#109938,62.8464445485378,0.127);
#6259=TOROIDAL_SURFACE('',#109948,59.0285554514622,0.127);
#6260=TOROIDAL_SURFACE('',#109982,62.8464445485378,0.127);
#6261=TOROIDAL_SURFACE('',#109992,59.0285554514622,0.127);
#6262=TOROIDAL_SURFACE('',#110026,62.8464445485378,0.127);
#6263=TOROIDAL_SURFACE('',#110036,59.0285554514622,0.127);
#6264=TOROIDAL_SURFACE('',#110070,62.8464445485378,0.127);
#6265=TOROIDAL_SURFACE('',#110080,59.0285554514622,0.127);
#6266=TOROIDAL_SURFACE('',#110114,62.8464445485378,0.127);
#6267=TOROIDAL_SURFACE('',#110124,59.0285554514622,0.127);
#6268=TOROIDAL_SURFACE('',#110158,62.8464445485378,0.127);
#6269=TOROIDAL_SURFACE('',#110168,59.0285554514622,0.127);
#6270=TOROIDAL_SURFACE('',#110185,65.381,0.127);
#6271=TOROIDAL_SURFACE('',#110189,68.623,0.127);
#6272=TOROIDAL_SURFACE('',#110193,68.877,0.127);
#6273=TOROIDAL_SURFACE('',#110207,65.0762,0.0762);
#6274=TOROIDAL_SURFACE('',#110211,65.1778,0.0762);
#6275=TOROIDAL_SURFACE('',#110221,71.3206076480316,0.8255);
#6276=TOROIDAL_SURFACE('',#110225,74.6340699810941,2.54);
#6277=TOROIDAL_SURFACE('',#110230,23.73,1.27);
#6278=TOROIDAL_SURFACE('',#110235,23.73,1.27);
#6279=TOROIDAL_SURFACE('',#110252,81.905,1.905);
#6280=TOROIDAL_SURFACE('',#110263,73.65,6.35);
#6281=TOROIDAL_SURFACE('',#110390,73.65,6.35);
#6282=TOROIDAL_SURFACE('',#110392,73.65,6.35);
#6283=TOROIDAL_SURFACE('',#110394,73.65,6.35);
#6284=TOROIDAL_SURFACE('',#110395,73.65,6.35);
#6285=TOROIDAL_SURFACE('',#110414,81.905,1.905);
#6286=TOROIDAL_SURFACE('',#110416,26.905,1.905);
#6287=TOROIDAL_SURFACE('',#110422,26.905,1.905);
#6288=TOROIDAL_SURFACE('',#110426,26.905,1.905);
#6289=TOROIDAL_SURFACE('',#110431,26.905,1.905);
#6290=TOROIDAL_SURFACE('',#110435,81.905,1.905);
#6291=TOROIDAL_SURFACE('',#110436,26.905,1.905);
#6292=TOROIDAL_SURFACE('',#110441,26.905,1.905);
#6293=TOROIDAL_SURFACE('',#110451,23.73,1.27);
#6294=TOROIDAL_SURFACE('',#110460,23.73,1.27);
#6295=TOROIDAL_SURFACE('',#110464,82.2472021719721,2.54);
#6296=TOROIDAL_SURFACE('',#110467,82.2472021719721,2.54);
#6297=TOROIDAL_SURFACE('',#110470,82.2472021719721,2.54);
#6298=TOROIDAL_SURFACE('',#110474,82.2472021719721,2.54);
#6299=TOROIDAL_SURFACE('',#110506,78.7299999999993,2.54);
#6300=TOROIDAL_SURFACE('',#110510,1.8415,0.0635);
#6301=TOROIDAL_SURFACE('',#110515,1.8415,0.0635);
#6302=TOROIDAL_SURFACE('',#110531,66.2265441972308,0.127);
#6303=TOROIDAL_SURFACE('',#110536,66.3535441972308,0.127);
#6304=TOROIDAL_SURFACE('',#110548,56.0881943187058,0.381);
#6305=TOROIDAL_SURFACE('',#110552,50.889,0.381);
#6306=TOROIDAL_SURFACE('',#110557,50.381,0.381);
#6307=TOROIDAL_SURFACE('',#110562,56.7377745952251,0.254);
#6308=TOROIDAL_SURFACE('',#110566,57.4087519663171,0.254);
#6309=TOROIDAL_SURFACE('',#110717,74.8702478255888,1.5875);
#6310=TOROIDAL_SURFACE('',#110799,23.73,0.762);
#6311=TOROIDAL_SURFACE('',#110806,23.73,0.762);
#6312=TOROIDAL_SURFACE('',#110808,23.73,0.762);
#6313=TOROIDAL_SURFACE('',#110814,23.73,0.762);
#6349=FACE_BOUND('',#13851,.T.);
#6350=FACE_BOUND('',#13857,.T.);
#6351=FACE_BOUND('',#13866,.T.);
#6352=FACE_BOUND('',#13886,.T.);
#6353=FACE_BOUND('',#13888,.T.);
#6354=FACE_BOUND('',#13892,.T.);
#6355=FACE_BOUND('',#13894,.T.);
#6356=FACE_BOUND('',#13898,.T.);
#6357=FACE_BOUND('',#13900,.T.);
#6358=FACE_BOUND('',#13904,.T.);
#6359=FACE_BOUND('',#13906,.T.);
#6360=FACE_BOUND('',#13912,.T.);
#6361=FACE_BOUND('',#13914,.T.);
#6362=FACE_BOUND('',#13920,.T.);
#6363=FACE_BOUND('',#13922,.T.);
#6364=FACE_BOUND('',#13926,.T.);
#6365=FACE_BOUND('',#13928,.T.);
#6366=FACE_BOUND('',#14475,.T.);
#6367=FACE_BOUND('',#14482,.T.);
#6368=FACE_BOUND('',#14484,.T.);
#6369=FACE_BOUND('',#17011,.T.);
#6370=FACE_BOUND('',#17018,.T.);
#6371=FACE_BOUND('',#17020,.T.);
#6372=FACE_BOUND('',#19008,.T.);
#6373=FACE_BOUND('',#19010,.T.);
#6374=FACE_BOUND('',#19012,.T.);
#6375=FACE_BOUND('',#19018,.T.);
#6376=FACE_BOUND('',#19020,.T.);
#6377=FACE_BOUND('',#19057,.T.);
#6378=FACE_BOUND('',#19067,.T.);
#6379=FACE_BOUND('',#19070,.T.);
#6380=FACE_BOUND('',#19073,.T.);
#6381=FACE_BOUND('',#19075,.T.);
#6382=FACE_BOUND('',#19088,.T.);
#6383=FACE_BOUND('',#19089,.T.);
#6384=FACE_BOUND('',#19090,.T.);
#6385=FACE_BOUND('',#19091,.T.);
#6386=FACE_BOUND('',#19092,.T.);
#6387=FACE_BOUND('',#19094,.T.);
#6388=FACE_BOUND('',#19096,.T.);
#6389=FACE_BOUND('',#19216,.T.);
#6390=FACE_BOUND('',#19222,.T.);
#6391=FACE_BOUND('',#19224,.T.);
#6392=FACE_BOUND('',#19226,.T.);
#6393=FACE_BOUND('',#19228,.T.);
#6394=FACE_BOUND('',#19241,.T.);
#6395=FACE_BOUND('',#19243,.T.);
#6396=FACE_BOUND('',#19245,.T.);
#6397=FACE_BOUND('',#19247,.T.);
#6398=FACE_BOUND('',#19249,.T.);
#6399=FACE_BOUND('',#19269,.T.);
#6400=FACE_BOUND('',#19305,.T.);
#6401=FACE_BOUND('',#19327,.T.);
#6402=FACE_BOUND('',#19331,.T.);
#6403=FACE_BOUND('',#19333,.T.);
#6404=FACE_BOUND('',#19335,.T.);
#6405=FACE_BOUND('',#19360,.T.);
#6406=FACE_BOUND('',#19361,.T.);
#6407=FACE_BOUND('',#19362,.T.);
#6408=FACE_BOUND('',#19363,.T.);
#6409=FACE_BOUND('',#19364,.T.);
#6410=FACE_BOUND('',#19366,.T.);
#6411=FACE_BOUND('',#19368,.T.);
#6412=FACE_BOUND('',#19370,.T.);
#6413=FACE_BOUND('',#19372,.T.);
#6414=FACE_BOUND('',#19374,.T.);
#6415=FACE_BOUND('',#19392,.T.);
#6416=FACE_BOUND('',#19393,.T.);
#6417=FACE_BOUND('',#19394,.T.);
#6418=FACE_BOUND('',#19395,.T.);
#6419=FACE_BOUND('',#19396,.T.);
#6420=FACE_BOUND('',#19399,.T.);
#6421=FACE_BOUND('',#19401,.T.);
#6422=FACE_BOUND('',#19403,.T.);
#6423=FACE_BOUND('',#19405,.T.);
#6424=FACE_BOUND('',#19410,.T.);
#6478=PLANE('',#98975);
#6479=PLANE('',#98976);
#6480=PLANE('',#98982);
#6481=PLANE('',#98983);
#6482=PLANE('',#98994);
#6483=PLANE('',#98995);
#6484=PLANE('',#98996);
#6485=PLANE('',#98997);
#6486=PLANE('',#98998);
#6487=PLANE('',#98999);
#6488=PLANE('',#99011);
#6489=PLANE('',#99012);
#6490=PLANE('',#99019);
#6491=PLANE('',#99020);
#6492=PLANE('',#99027);
#6493=PLANE('',#99028);
#6494=PLANE('',#99035);
#6495=PLANE('',#99036);
#6496=PLANE('',#99051);
#6497=PLANE('',#99052);
#6498=PLANE('',#99067);
#6499=PLANE('',#99068);
#6500=PLANE('',#99075);
#6501=PLANE('',#99076);
#6502=PLANE('',#99364);
#6503=PLANE('',#99371);
#6504=PLANE('',#99379);
#6505=PLANE('',#99393);
#6506=PLANE('',#99400);
#6507=PLANE('',#99408);
#6508=PLANE('',#99422);
#6509=PLANE('',#99429);
#6510=PLANE('',#99437);
#6511=PLANE('',#99451);
#6512=PLANE('',#99458);
#6513=PLANE('',#99466);
#6514=PLANE('',#99480);
#6515=PLANE('',#99487);
#6516=PLANE('',#99495);
#6517=PLANE('',#99509);
#6518=PLANE('',#99516);
#6519=PLANE('',#99524);
#6520=PLANE('',#99538);
#6521=PLANE('',#99545);
#6522=PLANE('',#99553);
#6523=PLANE('',#99567);
#6524=PLANE('',#99574);
#6525=PLANE('',#99582);
#6526=PLANE('',#99596);
#6527=PLANE('',#99603);
#6528=PLANE('',#99611);
#6529=PLANE('',#99625);
#6530=PLANE('',#99632);
#6531=PLANE('',#99640);
#6532=PLANE('',#99654);
#6533=PLANE('',#99661);
#6534=PLANE('',#99669);
#6535=PLANE('',#99683);
#6536=PLANE('',#99690);
#6537=PLANE('',#99698);
#6538=PLANE('',#99712);
#6539=PLANE('',#99719);
#6540=PLANE('',#99727);
#6541=PLANE('',#99741);
#6542=PLANE('',#99748);
#6543=PLANE('',#99756);
#6544=PLANE('',#99770);
#6545=PLANE('',#99777);
#6546=PLANE('',#99785);
#6547=PLANE('',#99799);
#6548=PLANE('',#99806);
#6549=PLANE('',#99814);
#6550=PLANE('',#99828);
#6551=PLANE('',#99835);
#6552=PLANE('',#99843);
#6553=PLANE('',#99857);
#6554=PLANE('',#99864);
#6555=PLANE('',#99872);
#6556=PLANE('',#99886);
#6557=PLANE('',#99893);
#6558=PLANE('',#99901);
#6559=PLANE('',#99915);
#6560=PLANE('',#99922);
#6561=PLANE('',#99930);
#6562=PLANE('',#99944);
#6563=PLANE('',#99951);
#6564=PLANE('',#99959);
#6565=PLANE('',#99973);
#6566=PLANE('',#99980);
#6567=PLANE('',#99988);
#6568=PLANE('',#100002);
#6569=PLANE('',#100009);
#6570=PLANE('',#100017);
#6571=PLANE('',#100031);
#6572=PLANE('',#100038);
#6573=PLANE('',#100046);
#6574=PLANE('',#100060);
#6575=PLANE('',#100067);
#6576=PLANE('',#100075);
#6577=PLANE('',#100089);
#6578=PLANE('',#100096);
#6579=PLANE('',#100104);
#6580=PLANE('',#100118);
#6581=PLANE('',#100125);
#6582=PLANE('',#100133);
#6583=PLANE('',#100147);
#6584=PLANE('',#100154);
#6585=PLANE('',#100162);
#6586=PLANE('',#100176);
#6587=PLANE('',#100183);
#6588=PLANE('',#100191);
#6589=PLANE('',#100205);
#6590=PLANE('',#100212);
#6591=PLANE('',#100220);
#6592=PLANE('',#100234);
#6593=PLANE('',#100241);
#6594=PLANE('',#100249);
#6595=PLANE('',#100263);
#6596=PLANE('',#100270);
#6597=PLANE('',#100278);
#6598=PLANE('',#100292);
#6599=PLANE('',#100299);
#6600=PLANE('',#100307);
#6601=PLANE('',#100321);
#6602=PLANE('',#100328);
#6603=PLANE('',#100336);
#6604=PLANE('',#100350);
#6605=PLANE('',#100357);
#6606=PLANE('',#100365);
#6607=PLANE('',#100379);
#6608=PLANE('',#100386);
#6609=PLANE('',#100394);
#6610=PLANE('',#100408);
#6611=PLANE('',#100415);
#6612=PLANE('',#100423);
#6613=PLANE('',#100437);
#6614=PLANE('',#100444);
#6615=PLANE('',#100452);
#6616=PLANE('',#100466);
#6617=PLANE('',#100473);
#6618=PLANE('',#100481);
#6619=PLANE('',#100495);
#6620=PLANE('',#100502);
#6621=PLANE('',#100510);
#6622=PLANE('',#100524);
#6623=PLANE('',#100531);
#6624=PLANE('',#100539);
#6625=PLANE('',#100553);
#6626=PLANE('',#100560);
#6627=PLANE('',#100568);
#6628=PLANE('',#100582);
#6629=PLANE('',#100589);
#6630=PLANE('',#100597);
#6631=PLANE('',#100611);
#6632=PLANE('',#100618);
#6633=PLANE('',#100626);
#6634=PLANE('',#100640);
#6635=PLANE('',#100647);
#6636=PLANE('',#100655);
#6637=PLANE('',#100669);
#6638=PLANE('',#100676);
#6639=PLANE('',#100684);
#6640=PLANE('',#100698);
#6641=PLANE('',#100705);
#6642=PLANE('',#100713);
#6643=PLANE('',#100727);
#6644=PLANE('',#100734);
#6645=PLANE('',#100742);
#6646=PLANE('',#100756);
#6647=PLANE('',#100763);
#6648=PLANE('',#100771);
#6649=PLANE('',#100785);
#6650=PLANE('',#100792);
#6651=PLANE('',#100800);
#6652=PLANE('',#100814);
#6653=PLANE('',#100821);
#6654=PLANE('',#100829);
#6655=PLANE('',#100843);
#6656=PLANE('',#100850);
#6657=PLANE('',#100858);
#6658=PLANE('',#100872);
#6659=PLANE('',#100879);
#6660=PLANE('',#100887);
#6661=PLANE('',#100901);
#6662=PLANE('',#100908);
#6663=PLANE('',#100916);
#6664=PLANE('',#100930);
#6665=PLANE('',#100937);
#6666=PLANE('',#100945);
#6667=PLANE('',#100959);
#6668=PLANE('',#100966);
#6669=PLANE('',#100974);
#6670=PLANE('',#100988);
#6671=PLANE('',#100995);
#6672=PLANE('',#101003);
#6673=PLANE('',#101017);
#6674=PLANE('',#101024);
#6675=PLANE('',#101032);
#6676=PLANE('',#101046);
#6677=PLANE('',#101053);
#6678=PLANE('',#101061);
#6679=PLANE('',#101075);
#6680=PLANE('',#101076);
#6681=PLANE('',#101083);
#6682=PLANE('',#101091);
#6683=PLANE('',#101093);
#6684=PLANE('',#101094);
#6685=PLANE('',#101107);
#6686=PLANE('',#101110);
#6687=PLANE('',#101115);
#6688=PLANE('',#101166);
#6689=PLANE('',#101169);
#6690=PLANE('',#101174);
#6691=PLANE('',#101179);
#6692=PLANE('',#101182);
#6693=PLANE('',#101187);
#6694=PLANE('',#101192);
#6695=PLANE('',#101195);
#6696=PLANE('',#101200);
#6697=PLANE('',#101205);
#6698=PLANE('',#101208);
#6699=PLANE('',#101213);
#6700=PLANE('',#101218);
#6701=PLANE('',#101221);
#6702=PLANE('',#101226);
#6703=PLANE('',#101231);
#6704=PLANE('',#101234);
#6705=PLANE('',#101239);
#6706=PLANE('',#101244);
#6707=PLANE('',#101247);
#6708=PLANE('',#101252);
#6709=PLANE('',#101257);
#6710=PLANE('',#101260);
#6711=PLANE('',#101265);
#6712=PLANE('',#101270);
#6713=PLANE('',#101273);
#6714=PLANE('',#101278);
#6715=PLANE('',#101283);
#6716=PLANE('',#101286);
#6717=PLANE('',#101291);
#6718=PLANE('',#101296);
#6719=PLANE('',#101299);
#6720=PLANE('',#101304);
#6721=PLANE('',#101309);
#6722=PLANE('',#101312);
#6723=PLANE('',#101317);
#6724=PLANE('',#101322);
#6725=PLANE('',#101325);
#6726=PLANE('',#101330);
#6727=PLANE('',#101335);
#6728=PLANE('',#101338);
#6729=PLANE('',#101343);
#6730=PLANE('',#101348);
#6731=PLANE('',#101351);
#6732=PLANE('',#101356);
#6733=PLANE('',#101361);
#6734=PLANE('',#101364);
#6735=PLANE('',#101369);
#6736=PLANE('',#101374);
#6737=PLANE('',#101377);
#6738=PLANE('',#101382);
#6739=PLANE('',#101387);
#6740=PLANE('',#101390);
#6741=PLANE('',#101395);
#6742=PLANE('',#101400);
#6743=PLANE('',#101403);
#6744=PLANE('',#101408);
#6745=PLANE('',#101413);
#6746=PLANE('',#101416);
#6747=PLANE('',#101421);
#6748=PLANE('',#101426);
#6749=PLANE('',#101429);
#6750=PLANE('',#101434);
#6751=PLANE('',#101439);
#6752=PLANE('',#101442);
#6753=PLANE('',#101447);
#6754=PLANE('',#101452);
#6755=PLANE('',#101455);
#6756=PLANE('',#101460);
#6757=PLANE('',#101465);
#6758=PLANE('',#101468);
#6759=PLANE('',#101473);
#6760=PLANE('',#101478);
#6761=PLANE('',#101481);
#6762=PLANE('',#101486);
#6763=PLANE('',#101491);
#6764=PLANE('',#101494);
#6765=PLANE('',#101499);
#6766=PLANE('',#101504);
#6767=PLANE('',#101507);
#6768=PLANE('',#101512);
#6769=PLANE('',#101517);
#6770=PLANE('',#101520);
#6771=PLANE('',#101525);
#6772=PLANE('',#101530);
#6773=PLANE('',#101533);
#6774=PLANE('',#101538);
#6775=PLANE('',#101543);
#6776=PLANE('',#101544);
#6777=PLANE('',#101549);
#6778=PLANE('',#101554);
#6779=PLANE('',#101557);
#6780=PLANE('',#101562);
#6781=PLANE('',#101567);
#6782=PLANE('',#101570);
#6783=PLANE('',#101575);
#6784=PLANE('',#101580);
#6785=PLANE('',#101583);
#6786=PLANE('',#101588);
#6787=PLANE('',#101593);
#6788=PLANE('',#101596);
#6789=PLANE('',#101601);
#6790=PLANE('',#101606);
#6791=PLANE('',#101609);
#6792=PLANE('',#101614);
#6793=PLANE('',#101619);
#6794=PLANE('',#101622);
#6795=PLANE('',#101627);
#6796=PLANE('',#101632);
#6797=PLANE('',#101635);
#6798=PLANE('',#101640);
#6799=PLANE('',#101645);
#6800=PLANE('',#101648);
#6801=PLANE('',#101653);
#6802=PLANE('',#101658);
#6803=PLANE('',#101661);
#6804=PLANE('',#101666);
#6805=PLANE('',#101671);
#6806=PLANE('',#101674);
#6807=PLANE('',#101679);
#6808=PLANE('',#101684);
#6809=PLANE('',#101687);
#6810=PLANE('',#101692);
#6811=PLANE('',#101697);
#6812=PLANE('',#101700);
#6813=PLANE('',#101705);
#6814=PLANE('',#101710);
#6815=PLANE('',#101713);
#6816=PLANE('',#101718);
#6817=PLANE('',#101723);
#6818=PLANE('',#101726);
#6819=PLANE('',#101731);
#6820=PLANE('',#101736);
#6821=PLANE('',#101737);
#6822=PLANE('',#101742);
#6823=PLANE('',#101747);
#6824=PLANE('',#101750);
#6825=PLANE('',#101755);
#6826=PLANE('',#101760);
#6827=PLANE('',#101763);
#6828=PLANE('',#101768);
#6829=PLANE('',#101773);
#6830=PLANE('',#101776);
#6831=PLANE('',#101781);
#6832=PLANE('',#101786);
#6833=PLANE('',#101789);
#6834=PLANE('',#101794);
#6835=PLANE('',#101799);
#6836=PLANE('',#101802);
#6837=PLANE('',#101807);
#6838=PLANE('',#101812);
#6839=PLANE('',#101815);
#6840=PLANE('',#101820);
#6841=PLANE('',#101825);
#6842=PLANE('',#101828);
#6843=PLANE('',#101833);
#6844=PLANE('',#101838);
#6845=PLANE('',#101841);
#6846=PLANE('',#101846);
#6847=PLANE('',#101851);
#6848=PLANE('',#101854);
#6849=PLANE('',#101859);
#6850=PLANE('',#101864);
#6851=PLANE('',#101867);
#6852=PLANE('',#101872);
#6853=PLANE('',#101877);
#6854=PLANE('',#101880);
#6855=PLANE('',#101885);
#6856=PLANE('',#101890);
#6857=PLANE('',#101893);
#6858=PLANE('',#101898);
#6859=PLANE('',#101903);
#6860=PLANE('',#101906);
#6861=PLANE('',#101911);
#6862=PLANE('',#101916);
#6863=PLANE('',#101919);
#6864=PLANE('',#101924);
#6865=PLANE('',#104918);
#6866=PLANE('',#104925);
#6867=PLANE('',#104933);
#6868=PLANE('',#104947);
#6869=PLANE('',#104954);
#6870=PLANE('',#104962);
#6871=PLANE('',#104976);
#6872=PLANE('',#104983);
#6873=PLANE('',#104991);
#6874=PLANE('',#105005);
#6875=PLANE('',#105012);
#6876=PLANE('',#105020);
#6877=PLANE('',#105034);
#6878=PLANE('',#105041);
#6879=PLANE('',#105049);
#6880=PLANE('',#105063);
#6881=PLANE('',#105070);
#6882=PLANE('',#105078);
#6883=PLANE('',#105092);
#6884=PLANE('',#105099);
#6885=PLANE('',#105107);
#6886=PLANE('',#105121);
#6887=PLANE('',#105128);
#6888=PLANE('',#105136);
#6889=PLANE('',#105150);
#6890=PLANE('',#105157);
#6891=PLANE('',#105165);
#6892=PLANE('',#105179);
#6893=PLANE('',#105186);
#6894=PLANE('',#105194);
#6895=PLANE('',#105208);
#6896=PLANE('',#105215);
#6897=PLANE('',#105223);
#6898=PLANE('',#105237);
#6899=PLANE('',#105244);
#6900=PLANE('',#105252);
#6901=PLANE('',#105266);
#6902=PLANE('',#105273);
#6903=PLANE('',#105281);
#6904=PLANE('',#105295);
#6905=PLANE('',#105302);
#6906=PLANE('',#105310);
#6907=PLANE('',#105324);
#6908=PLANE('',#105331);
#6909=PLANE('',#105339);
#6910=PLANE('',#105353);
#6911=PLANE('',#105360);
#6912=PLANE('',#105368);
#6913=PLANE('',#105382);
#6914=PLANE('',#105389);
#6915=PLANE('',#105397);
#6916=PLANE('',#105411);
#6917=PLANE('',#105418);
#6918=PLANE('',#105426);
#6919=PLANE('',#105440);
#6920=PLANE('',#105447);
#6921=PLANE('',#105455);
#6922=PLANE('',#105469);
#6923=PLANE('',#105476);
#6924=PLANE('',#105484);
#6925=PLANE('',#105498);
#6926=PLANE('',#105505);
#6927=PLANE('',#105513);
#6928=PLANE('',#105527);
#6929=PLANE('',#105534);
#6930=PLANE('',#105542);
#6931=PLANE('',#105556);
#6932=PLANE('',#105563);
#6933=PLANE('',#105571);
#6934=PLANE('',#105585);
#6935=PLANE('',#105592);
#6936=PLANE('',#105600);
#6937=PLANE('',#105614);
#6938=PLANE('',#105621);
#6939=PLANE('',#105629);
#6940=PLANE('',#105643);
#6941=PLANE('',#105650);
#6942=PLANE('',#105658);
#6943=PLANE('',#105672);
#6944=PLANE('',#105679);
#6945=PLANE('',#105687);
#6946=PLANE('',#105701);
#6947=PLANE('',#105708);
#6948=PLANE('',#105716);
#6949=PLANE('',#105730);
#6950=PLANE('',#105737);
#6951=PLANE('',#105745);
#6952=PLANE('',#105759);
#6953=PLANE('',#105766);
#6954=PLANE('',#105774);
#6955=PLANE('',#105788);
#6956=PLANE('',#105795);
#6957=PLANE('',#105803);
#6958=PLANE('',#105817);
#6959=PLANE('',#105824);
#6960=PLANE('',#105832);
#6961=PLANE('',#105846);
#6962=PLANE('',#105853);
#6963=PLANE('',#105861);
#6964=PLANE('',#105875);
#6965=PLANE('',#105882);
#6966=PLANE('',#105890);
#6967=PLANE('',#105904);
#6968=PLANE('',#105911);
#6969=PLANE('',#105919);
#6970=PLANE('',#105933);
#6971=PLANE('',#105940);
#6972=PLANE('',#105948);
#6973=PLANE('',#105962);
#6974=PLANE('',#105969);
#6975=PLANE('',#105977);
#6976=PLANE('',#105991);
#6977=PLANE('',#105998);
#6978=PLANE('',#106006);
#6979=PLANE('',#106020);
#6980=PLANE('',#106027);
#6981=PLANE('',#106035);
#6982=PLANE('',#106049);
#6983=PLANE('',#106056);
#6984=PLANE('',#106064);
#6985=PLANE('',#106078);
#6986=PLANE('',#106085);
#6987=PLANE('',#106093);
#6988=PLANE('',#106107);
#6989=PLANE('',#106114);
#6990=PLANE('',#106122);
#6991=PLANE('',#106136);
#6992=PLANE('',#106143);
#6993=PLANE('',#106151);
#6994=PLANE('',#106165);
#6995=PLANE('',#106172);
#6996=PLANE('',#106180);
#6997=PLANE('',#106194);
#6998=PLANE('',#106201);
#6999=PLANE('',#106209);
#7000=PLANE('',#106223);
#7001=PLANE('',#106230);
#7002=PLANE('',#106238);
#7003=PLANE('',#106252);
#7004=PLANE('',#106259);
#7005=PLANE('',#106267);
#7006=PLANE('',#106281);
#7007=PLANE('',#106288);
#7008=PLANE('',#106296);
#7009=PLANE('',#106310);
#7010=PLANE('',#106317);
#7011=PLANE('',#106325);
#7012=PLANE('',#106339);
#7013=PLANE('',#106346);
#7014=PLANE('',#106354);
#7015=PLANE('',#106368);
#7016=PLANE('',#106375);
#7017=PLANE('',#106383);
#7018=PLANE('',#106397);
#7019=PLANE('',#106404);
#7020=PLANE('',#106412);
#7021=PLANE('',#106426);
#7022=PLANE('',#106433);
#7023=PLANE('',#106441);
#7024=PLANE('',#106455);
#7025=PLANE('',#106462);
#7026=PLANE('',#106470);
#7027=PLANE('',#106484);
#7028=PLANE('',#106491);
#7029=PLANE('',#106499);
#7030=PLANE('',#106513);
#7031=PLANE('',#106520);
#7032=PLANE('',#106528);
#7033=PLANE('',#106542);
#7034=PLANE('',#106549);
#7035=PLANE('',#106557);
#7036=PLANE('',#106571);
#7037=PLANE('',#106578);
#7038=PLANE('',#106586);
#7039=PLANE('',#106600);
#7040=PLANE('',#106607);
#7041=PLANE('',#106615);
#7042=PLANE('',#106629);
#7043=PLANE('',#106630);
#7044=PLANE('',#106637);
#7045=PLANE('',#106645);
#7046=PLANE('',#106647);
#7047=PLANE('',#106648);
#7048=PLANE('',#106661);
#7049=PLANE('',#106664);
#7050=PLANE('',#106669);
#7051=PLANE('',#106720);
#7052=PLANE('',#106723);
#7053=PLANE('',#106728);
#7054=PLANE('',#106733);
#7055=PLANE('',#106736);
#7056=PLANE('',#106741);
#7057=PLANE('',#106746);
#7058=PLANE('',#106749);
#7059=PLANE('',#106754);
#7060=PLANE('',#106759);
#7061=PLANE('',#106762);
#7062=PLANE('',#106767);
#7063=PLANE('',#106772);
#7064=PLANE('',#106775);
#7065=PLANE('',#106780);
#7066=PLANE('',#106785);
#7067=PLANE('',#106788);
#7068=PLANE('',#106793);
#7069=PLANE('',#106798);
#7070=PLANE('',#106801);
#7071=PLANE('',#106806);
#7072=PLANE('',#106811);
#7073=PLANE('',#106814);
#7074=PLANE('',#106819);
#7075=PLANE('',#106824);
#7076=PLANE('',#106827);
#7077=PLANE('',#106832);
#7078=PLANE('',#106837);
#7079=PLANE('',#106840);
#7080=PLANE('',#106845);
#7081=PLANE('',#106850);
#7082=PLANE('',#106853);
#7083=PLANE('',#106858);
#7084=PLANE('',#106863);
#7085=PLANE('',#106866);
#7086=PLANE('',#106871);
#7087=PLANE('',#106876);
#7088=PLANE('',#106879);
#7089=PLANE('',#106884);
#7090=PLANE('',#106889);
#7091=PLANE('',#106892);
#7092=PLANE('',#106897);
#7093=PLANE('',#106902);
#7094=PLANE('',#106905);
#7095=PLANE('',#106910);
#7096=PLANE('',#106915);
#7097=PLANE('',#106918);
#7098=PLANE('',#106923);
#7099=PLANE('',#106928);
#7100=PLANE('',#106931);
#7101=PLANE('',#106936);
#7102=PLANE('',#106941);
#7103=PLANE('',#106944);
#7104=PLANE('',#106949);
#7105=PLANE('',#106954);
#7106=PLANE('',#106957);
#7107=PLANE('',#106962);
#7108=PLANE('',#106967);
#7109=PLANE('',#106970);
#7110=PLANE('',#106975);
#7111=PLANE('',#106980);
#7112=PLANE('',#106983);
#7113=PLANE('',#106988);
#7114=PLANE('',#106993);
#7115=PLANE('',#106996);
#7116=PLANE('',#107001);
#7117=PLANE('',#107006);
#7118=PLANE('',#107009);
#7119=PLANE('',#107014);
#7120=PLANE('',#107019);
#7121=PLANE('',#107022);
#7122=PLANE('',#107027);
#7123=PLANE('',#107032);
#7124=PLANE('',#107035);
#7125=PLANE('',#107040);
#7126=PLANE('',#107045);
#7127=PLANE('',#107048);
#7128=PLANE('',#107053);
#7129=PLANE('',#107058);
#7130=PLANE('',#107061);
#7131=PLANE('',#107066);
#7132=PLANE('',#107071);
#7133=PLANE('',#107074);
#7134=PLANE('',#107079);
#7135=PLANE('',#107084);
#7136=PLANE('',#107087);
#7137=PLANE('',#107092);
#7138=PLANE('',#107097);
#7139=PLANE('',#107098);
#7140=PLANE('',#107103);
#7141=PLANE('',#107108);
#7142=PLANE('',#107111);
#7143=PLANE('',#107116);
#7144=PLANE('',#107121);
#7145=PLANE('',#107124);
#7146=PLANE('',#107129);
#7147=PLANE('',#107134);
#7148=PLANE('',#107137);
#7149=PLANE('',#107142);
#7150=PLANE('',#107147);
#7151=PLANE('',#107150);
#7152=PLANE('',#107155);
#7153=PLANE('',#107160);
#7154=PLANE('',#107163);
#7155=PLANE('',#107168);
#7156=PLANE('',#107173);
#7157=PLANE('',#107176);
#7158=PLANE('',#107181);
#7159=PLANE('',#107186);
#7160=PLANE('',#107189);
#7161=PLANE('',#107194);
#7162=PLANE('',#107199);
#7163=PLANE('',#107202);
#7164=PLANE('',#107207);
#7165=PLANE('',#107212);
#7166=PLANE('',#107215);
#7167=PLANE('',#107220);
#7168=PLANE('',#107225);
#7169=PLANE('',#107228);
#7170=PLANE('',#107233);
#7171=PLANE('',#107238);
#7172=PLANE('',#107241);
#7173=PLANE('',#107246);
#7174=PLANE('',#107251);
#7175=PLANE('',#107254);
#7176=PLANE('',#107259);
#7177=PLANE('',#107264);
#7178=PLANE('',#107267);
#7179=PLANE('',#107272);
#7180=PLANE('',#107277);
#7181=PLANE('',#107280);
#7182=PLANE('',#107285);
#7183=PLANE('',#107290);
#7184=PLANE('',#107291);
#7185=PLANE('',#107296);
#7186=PLANE('',#107301);
#7187=PLANE('',#107304);
#7188=PLANE('',#107309);
#7189=PLANE('',#107314);
#7190=PLANE('',#107317);
#7191=PLANE('',#107322);
#7192=PLANE('',#107327);
#7193=PLANE('',#107330);
#7194=PLANE('',#107335);
#7195=PLANE('',#107340);
#7196=PLANE('',#107343);
#7197=PLANE('',#107348);
#7198=PLANE('',#107353);
#7199=PLANE('',#107356);
#7200=PLANE('',#107361);
#7201=PLANE('',#107366);
#7202=PLANE('',#107369);
#7203=PLANE('',#107374);
#7204=PLANE('',#107379);
#7205=PLANE('',#107382);
#7206=PLANE('',#107387);
#7207=PLANE('',#107392);
#7208=PLANE('',#107395);
#7209=PLANE('',#107400);
#7210=PLANE('',#107405);
#7211=PLANE('',#107408);
#7212=PLANE('',#107413);
#7213=PLANE('',#107418);
#7214=PLANE('',#107421);
#7215=PLANE('',#107426);
#7216=PLANE('',#107431);
#7217=PLANE('',#107434);
#7218=PLANE('',#107439);
#7219=PLANE('',#107444);
#7220=PLANE('',#107447);
#7221=PLANE('',#107452);
#7222=PLANE('',#107457);
#7223=PLANE('',#107460);
#7224=PLANE('',#107465);
#7225=PLANE('',#107470);
#7226=PLANE('',#107473);
#7227=PLANE('',#107478);
#7228=PLANE('',#110204);
#7229=PLANE('',#110205);
#7230=PLANE('',#110206);
#7231=PLANE('',#110219);
#7232=PLANE('',#110220);
#7233=PLANE('',#110302);
#7234=PLANE('',#110303);
#7235=PLANE('',#110304);
#7236=PLANE('',#110313);
#7237=PLANE('',#110317);
#7238=PLANE('',#110321);
#7239=PLANE('',#110325);
#7240=PLANE('',#110329);
#7241=PLANE('',#110330);
#7242=PLANE('',#110332);
#7243=PLANE('',#110334);
#7244=PLANE('',#110341);
#7245=PLANE('',#110344);
#7246=PLANE('',#110350);
#7247=PLANE('',#110355);
#7248=PLANE('',#110361);
#7249=PLANE('',#110363);
#7250=PLANE('',#110365);
#7251=PLANE('',#110366);
#7252=PLANE('',#110367);
#7253=PLANE('',#110368);
#7254=PLANE('',#110372);
#7255=PLANE('',#110373);
#7256=PLANE('',#110374);
#7257=PLANE('',#110380);
#7258=PLANE('',#110381);
#7259=PLANE('',#110382);
#7260=PLANE('',#110385);
#7261=PLANE('',#110387);
#7262=PLANE('',#110388);
#7263=PLANE('',#110389);
#7264=PLANE('',#110530);
#7265=PLANE('',#110546);
#7266=PLANE('',#110547);
#7267=PLANE('',#110582);
#7268=PLANE('',#110583);
#7269=PLANE('',#110584);
#7270=PLANE('',#110585);
#7271=PLANE('',#110586);
#7272=PLANE('',#110617);
#7273=PLANE('',#110618);
#7274=PLANE('',#110631);
#7275=PLANE('',#110632);
#7276=PLANE('',#110633);
#7277=PLANE('',#110634);
#7278=PLANE('',#110635);
#7279=PLANE('',#110636);
#7280=PLANE('',#110637);
#7281=PLANE('',#110669);
#7282=PLANE('',#110670);
#7283=PLANE('',#110683);
#7284=PLANE('',#110684);
#7285=PLANE('',#110685);
#7286=PLANE('',#110686);
#7287=PLANE('',#110687);
#7288=PLANE('',#110688);
#7289=PLANE('',#110689);
#7290=PLANE('',#110709);
#7291=PLANE('',#110710);
#7292=PLANE('',#110760);
#7293=PLANE('',#110764);
#7294=PLANE('',#110768);
#7295=PLANE('',#110772);
#7296=PLANE('',#110773);
#7297=PLANE('',#110778);
#7298=PLANE('',#110779);
#7299=PLANE('',#110780);
#7300=PLANE('',#110781);
#7301=PLANE('',#110782);
#7302=PLANE('',#110789);
#7303=PLANE('',#110792);
#7304=PLANE('',#110795);
#7305=PLANE('',#110798);
#7306=PLANE('',#110815);
#7307=PLANE('',#110819);
#7308=PLANE('',#110822);
#7309=PLANE('',#110823);
#7310=PLANE('',#110824);
#7311=PLANE('',#110827);
#7312=PLANE('',#110828);
#7313=PLANE('',#110829);
#7314=PLANE('',#110832);
#7315=PLANE('',#110833);
#7707=FACE_OUTER_BOUND('',#13844,.T.);
#7708=FACE_OUTER_BOUND('',#13845,.T.);
#7709=FACE_OUTER_BOUND('',#13846,.T.);
#7710=FACE_OUTER_BOUND('',#13847,.T.);
#7711=FACE_OUTER_BOUND('',#13848,.T.);
#7712=FACE_OUTER_BOUND('',#13849,.T.);
#7713=FACE_OUTER_BOUND('',#13850,.T.);
#7714=FACE_OUTER_BOUND('',#13852,.T.);
#7715=FACE_OUTER_BOUND('',#13853,.T.);
#7716=FACE_OUTER_BOUND('',#13854,.T.);
#7717=FACE_OUTER_BOUND('',#13855,.T.);
#7718=FACE_OUTER_BOUND('',#13856,.T.);
#7719=FACE_OUTER_BOUND('',#13858,.T.);
#7720=FACE_OUTER_BOUND('',#13859,.T.);
#7721=FACE_OUTER_BOUND('',#13860,.T.);
#7722=FACE_OUTER_BOUND('',#13861,.T.);
#7723=FACE_OUTER_BOUND('',#13862,.T.);
#7724=FACE_OUTER_BOUND('',#13863,.T.);
#7725=FACE_OUTER_BOUND('',#13864,.T.);
#7726=FACE_OUTER_BOUND('',#13865,.T.);
#7727=FACE_OUTER_BOUND('',#13867,.T.);
#7728=FACE_OUTER_BOUND('',#13868,.T.);
#7729=FACE_OUTER_BOUND('',#13869,.T.);
#7730=FACE_OUTER_BOUND('',#13870,.T.);
#7731=FACE_OUTER_BOUND('',#13871,.T.);
#7732=FACE_OUTER_BOUND('',#13872,.T.);
#7733=FACE_OUTER_BOUND('',#13873,.T.);
#7734=FACE_OUTER_BOUND('',#13874,.T.);
#7735=FACE_OUTER_BOUND('',#13875,.T.);
#7736=FACE_OUTER_BOUND('',#13876,.T.);
#7737=FACE_OUTER_BOUND('',#13877,.T.);
#7738=FACE_OUTER_BOUND('',#13878,.T.);
#7739=FACE_OUTER_BOUND('',#13879,.T.);
#7740=FACE_OUTER_BOUND('',#13880,.T.);
#7741=FACE_OUTER_BOUND('',#13881,.T.);
#7742=FACE_OUTER_BOUND('',#13882,.T.);
#7743=FACE_OUTER_BOUND('',#13883,.T.);
#7744=FACE_OUTER_BOUND('',#13884,.T.);
#7745=FACE_OUTER_BOUND('',#13885,.T.);
#7746=FACE_OUTER_BOUND('',#13887,.T.);
#7747=FACE_OUTER_BOUND('',#13889,.T.);
#7748=FACE_OUTER_BOUND('',#13890,.T.);
#7749=FACE_OUTER_BOUND('',#13891,.T.);
#7750=FACE_OUTER_BOUND('',#13893,.T.);
#7751=FACE_OUTER_BOUND('',#13895,.T.);
#7752=FACE_OUTER_BOUND('',#13896,.T.);
#7753=FACE_OUTER_BOUND('',#13897,.T.);
#7754=FACE_OUTER_BOUND('',#13899,.T.);
#7755=FACE_OUTER_BOUND('',#13901,.T.);
#7756=FACE_OUTER_BOUND('',#13902,.T.);
#7757=FACE_OUTER_BOUND('',#13903,.T.);
#7758=FACE_OUTER_BOUND('',#13905,.T.);
#7759=FACE_OUTER_BOUND('',#13907,.T.);
#7760=FACE_OUTER_BOUND('',#13908,.T.);
#7761=FACE_OUTER_BOUND('',#13909,.T.);
#7762=FACE_OUTER_BOUND('',#13910,.T.);
#7763=FACE_OUTER_BOUND('',#13911,.T.);
#7764=FACE_OUTER_BOUND('',#13913,.T.);
#7765=FACE_OUTER_BOUND('',#13915,.T.);
#7766=FACE_OUTER_BOUND('',#13916,.T.);
#7767=FACE_OUTER_BOUND('',#13917,.T.);
#7768=FACE_OUTER_BOUND('',#13918,.T.);
#7769=FACE_OUTER_BOUND('',#13919,.T.);
#7770=FACE_OUTER_BOUND('',#13921,.T.);
#7771=FACE_OUTER_BOUND('',#13923,.T.);
#7772=FACE_OUTER_BOUND('',#13924,.T.);
#7773=FACE_OUTER_BOUND('',#13925,.T.);
#7774=FACE_OUTER_BOUND('',#13927,.T.);
#7775=FACE_OUTER_BOUND('',#13929,.T.);
#7776=FACE_OUTER_BOUND('',#13930,.T.);
#7777=FACE_OUTER_BOUND('',#13931,.T.);
#7778=FACE_OUTER_BOUND('',#13932,.T.);
#7779=FACE_OUTER_BOUND('',#13933,.T.);
#7780=FACE_OUTER_BOUND('',#13934,.T.);
#7781=FACE_OUTER_BOUND('',#13935,.T.);
#7782=FACE_OUTER_BOUND('',#13936,.T.);
#7783=FACE_OUTER_BOUND('',#13937,.T.);
#7784=FACE_OUTER_BOUND('',#13938,.T.);
#7785=FACE_OUTER_BOUND('',#13939,.T.);
#7786=FACE_OUTER_BOUND('',#13940,.T.);
#7787=FACE_OUTER_BOUND('',#13941,.T.);
#7788=FACE_OUTER_BOUND('',#13942,.T.);
#7789=FACE_OUTER_BOUND('',#13943,.T.);
#7790=FACE_OUTER_BOUND('',#13944,.T.);
#7791=FACE_OUTER_BOUND('',#13945,.T.);
#7792=FACE_OUTER_BOUND('',#13946,.T.);
#7793=FACE_OUTER_BOUND('',#13947,.T.);
#7794=FACE_OUTER_BOUND('',#13948,.T.);
#7795=FACE_OUTER_BOUND('',#13949,.T.);
#7796=FACE_OUTER_BOUND('',#13950,.T.);
#7797=FACE_OUTER_BOUND('',#13951,.T.);
#7798=FACE_OUTER_BOUND('',#13952,.T.);
#7799=FACE_OUTER_BOUND('',#13953,.T.);
#7800=FACE_OUTER_BOUND('',#13954,.T.);
#7801=FACE_OUTER_BOUND('',#13955,.T.);
#7802=FACE_OUTER_BOUND('',#13956,.T.);
#7803=FACE_OUTER_BOUND('',#13957,.T.);
#7804=FACE_OUTER_BOUND('',#13958,.T.);
#7805=FACE_OUTER_BOUND('',#13959,.T.);
#7806=FACE_OUTER_BOUND('',#13960,.T.);
#7807=FACE_OUTER_BOUND('',#13961,.T.);
#7808=FACE_OUTER_BOUND('',#13962,.T.);
#7809=FACE_OUTER_BOUND('',#13963,.T.);
#7810=FACE_OUTER_BOUND('',#13964,.T.);
#7811=FACE_OUTER_BOUND('',#13965,.T.);
#7812=FACE_OUTER_BOUND('',#13966,.T.);
#7813=FACE_OUTER_BOUND('',#13967,.T.);
#7814=FACE_OUTER_BOUND('',#13968,.T.);
#7815=FACE_OUTER_BOUND('',#13969,.T.);
#7816=FACE_OUTER_BOUND('',#13970,.T.);
#7817=FACE_OUTER_BOUND('',#13971,.T.);
#7818=FACE_OUTER_BOUND('',#13972,.T.);
#7819=FACE_OUTER_BOUND('',#13973,.T.);
#7820=FACE_OUTER_BOUND('',#13974,.T.);
#7821=FACE_OUTER_BOUND('',#13975,.T.);
#7822=FACE_OUTER_BOUND('',#13976,.T.);
#7823=FACE_OUTER_BOUND('',#13977,.T.);
#7824=FACE_OUTER_BOUND('',#13978,.T.);
#7825=FACE_OUTER_BOUND('',#13979,.T.);
#7826=FACE_OUTER_BOUND('',#13980,.T.);
#7827=FACE_OUTER_BOUND('',#13981,.T.);
#7828=FACE_OUTER_BOUND('',#13982,.T.);
#7829=FACE_OUTER_BOUND('',#13983,.T.);
#7830=FACE_OUTER_BOUND('',#13984,.T.);
#7831=FACE_OUTER_BOUND('',#13985,.T.);
#7832=FACE_OUTER_BOUND('',#13986,.T.);
#7833=FACE_OUTER_BOUND('',#13987,.T.);
#7834=FACE_OUTER_BOUND('',#13988,.T.);
#7835=FACE_OUTER_BOUND('',#13989,.T.);
#7836=FACE_OUTER_BOUND('',#13990,.T.);
#7837=FACE_OUTER_BOUND('',#13991,.T.);
#7838=FACE_OUTER_BOUND('',#13992,.T.);
#7839=FACE_OUTER_BOUND('',#13993,.T.);
#7840=FACE_OUTER_BOUND('',#13994,.T.);
#7841=FACE_OUTER_BOUND('',#13995,.T.);
#7842=FACE_OUTER_BOUND('',#13996,.T.);
#7843=FACE_OUTER_BOUND('',#13997,.T.);
#7844=FACE_OUTER_BOUND('',#13998,.T.);
#7845=FACE_OUTER_BOUND('',#13999,.T.);
#7846=FACE_OUTER_BOUND('',#14000,.T.);
#7847=FACE_OUTER_BOUND('',#14001,.T.);
#7848=FACE_OUTER_BOUND('',#14002,.T.);
#7849=FACE_OUTER_BOUND('',#14003,.T.);
#7850=FACE_OUTER_BOUND('',#14004,.T.);
#7851=FACE_OUTER_BOUND('',#14005,.T.);
#7852=FACE_OUTER_BOUND('',#14006,.T.);
#7853=FACE_OUTER_BOUND('',#14007,.T.);
#7854=FACE_OUTER_BOUND('',#14008,.T.);
#7855=FACE_OUTER_BOUND('',#14009,.T.);
#7856=FACE_OUTER_BOUND('',#14010,.T.);
#7857=FACE_OUTER_BOUND('',#14011,.T.);
#7858=FACE_OUTER_BOUND('',#14012,.T.);
#7859=FACE_OUTER_BOUND('',#14013,.T.);
#7860=FACE_OUTER_BOUND('',#14014,.T.);
#7861=FACE_OUTER_BOUND('',#14015,.T.);
#7862=FACE_OUTER_BOUND('',#14016,.T.);
#7863=FACE_OUTER_BOUND('',#14017,.T.);
#7864=FACE_OUTER_BOUND('',#14018,.T.);
#7865=FACE_OUTER_BOUND('',#14019,.T.);
#7866=FACE_OUTER_BOUND('',#14020,.T.);
#7867=FACE_OUTER_BOUND('',#14021,.T.);
#7868=FACE_OUTER_BOUND('',#14022,.T.);
#7869=FACE_OUTER_BOUND('',#14023,.T.);
#7870=FACE_OUTER_BOUND('',#14024,.T.);
#7871=FACE_OUTER_BOUND('',#14025,.T.);
#7872=FACE_OUTER_BOUND('',#14026,.T.);
#7873=FACE_OUTER_BOUND('',#14027,.T.);
#7874=FACE_OUTER_BOUND('',#14028,.T.);
#7875=FACE_OUTER_BOUND('',#14029,.T.);
#7876=FACE_OUTER_BOUND('',#14030,.T.);
#7877=FACE_OUTER_BOUND('',#14031,.T.);
#7878=FACE_OUTER_BOUND('',#14032,.T.);
#7879=FACE_OUTER_BOUND('',#14033,.T.);
#7880=FACE_OUTER_BOUND('',#14034,.T.);
#7881=FACE_OUTER_BOUND('',#14035,.T.);
#7882=FACE_OUTER_BOUND('',#14036,.T.);
#7883=FACE_OUTER_BOUND('',#14037,.T.);
#7884=FACE_OUTER_BOUND('',#14038,.T.);
#7885=FACE_OUTER_BOUND('',#14039,.T.);
#7886=FACE_OUTER_BOUND('',#14040,.T.);
#7887=FACE_OUTER_BOUND('',#14041,.T.);
#7888=FACE_OUTER_BOUND('',#14042,.T.);
#7889=FACE_OUTER_BOUND('',#14043,.T.);
#7890=FACE_OUTER_BOUND('',#14044,.T.);
#7891=FACE_OUTER_BOUND('',#14045,.T.);
#7892=FACE_OUTER_BOUND('',#14046,.T.);
#7893=FACE_OUTER_BOUND('',#14047,.T.);
#7894=FACE_OUTER_BOUND('',#14048,.T.);
#7895=FACE_OUTER_BOUND('',#14049,.T.);
#7896=FACE_OUTER_BOUND('',#14050,.T.);
#7897=FACE_OUTER_BOUND('',#14051,.T.);
#7898=FACE_OUTER_BOUND('',#14052,.T.);
#7899=FACE_OUTER_BOUND('',#14053,.T.);
#7900=FACE_OUTER_BOUND('',#14054,.T.);
#7901=FACE_OUTER_BOUND('',#14055,.T.);
#7902=FACE_OUTER_BOUND('',#14056,.T.);
#7903=FACE_OUTER_BOUND('',#14057,.T.);
#7904=FACE_OUTER_BOUND('',#14058,.T.);
#7905=FACE_OUTER_BOUND('',#14059,.T.);
#7906=FACE_OUTER_BOUND('',#14060,.T.);
#7907=FACE_OUTER_BOUND('',#14061,.T.);
#7908=FACE_OUTER_BOUND('',#14062,.T.);
#7909=FACE_OUTER_BOUND('',#14063,.T.);
#7910=FACE_OUTER_BOUND('',#14064,.T.);
#7911=FACE_OUTER_BOUND('',#14065,.T.);
#7912=FACE_OUTER_BOUND('',#14066,.T.);
#7913=FACE_OUTER_BOUND('',#14067,.T.);
#7914=FACE_OUTER_BOUND('',#14068,.T.);
#7915=FACE_OUTER_BOUND('',#14069,.T.);
#7916=FACE_OUTER_BOUND('',#14070,.T.);
#7917=FACE_OUTER_BOUND('',#14071,.T.);
#7918=FACE_OUTER_BOUND('',#14072,.T.);
#7919=FACE_OUTER_BOUND('',#14073,.T.);
#7920=FACE_OUTER_BOUND('',#14074,.T.);
#7921=FACE_OUTER_BOUND('',#14075,.T.);
#7922=FACE_OUTER_BOUND('',#14076,.T.);
#7923=FACE_OUTER_BOUND('',#14077,.T.);
#7924=FACE_OUTER_BOUND('',#14078,.T.);
#7925=FACE_OUTER_BOUND('',#14079,.T.);
#7926=FACE_OUTER_BOUND('',#14080,.T.);
#7927=FACE_OUTER_BOUND('',#14081,.T.);
#7928=FACE_OUTER_BOUND('',#14082,.T.);
#7929=FACE_OUTER_BOUND('',#14083,.T.);
#7930=FACE_OUTER_BOUND('',#14084,.T.);
#7931=FACE_OUTER_BOUND('',#14085,.T.);
#7932=FACE_OUTER_BOUND('',#14086,.T.);
#7933=FACE_OUTER_BOUND('',#14087,.T.);
#7934=FACE_OUTER_BOUND('',#14088,.T.);
#7935=FACE_OUTER_BOUND('',#14089,.T.);
#7936=FACE_OUTER_BOUND('',#14090,.T.);
#7937=FACE_OUTER_BOUND('',#14091,.T.);
#7938=FACE_OUTER_BOUND('',#14092,.T.);
#7939=FACE_OUTER_BOUND('',#14093,.T.);
#7940=FACE_OUTER_BOUND('',#14094,.T.);
#7941=FACE_OUTER_BOUND('',#14095,.T.);
#7942=FACE_OUTER_BOUND('',#14096,.T.);
#7943=FACE_OUTER_BOUND('',#14097,.T.);
#7944=FACE_OUTER_BOUND('',#14098,.T.);
#7945=FACE_OUTER_BOUND('',#14099,.T.);
#7946=FACE_OUTER_BOUND('',#14100,.T.);
#7947=FACE_OUTER_BOUND('',#14101,.T.);
#7948=FACE_OUTER_BOUND('',#14102,.T.);
#7949=FACE_OUTER_BOUND('',#14103,.T.);
#7950=FACE_OUTER_BOUND('',#14104,.T.);
#7951=FACE_OUTER_BOUND('',#14105,.T.);
#7952=FACE_OUTER_BOUND('',#14106,.T.);
#7953=FACE_OUTER_BOUND('',#14107,.T.);
#7954=FACE_OUTER_BOUND('',#14108,.T.);
#7955=FACE_OUTER_BOUND('',#14109,.T.);
#7956=FACE_OUTER_BOUND('',#14110,.T.);
#7957=FACE_OUTER_BOUND('',#14111,.T.);
#7958=FACE_OUTER_BOUND('',#14112,.T.);
#7959=FACE_OUTER_BOUND('',#14113,.T.);
#7960=FACE_OUTER_BOUND('',#14114,.T.);
#7961=FACE_OUTER_BOUND('',#14115,.T.);
#7962=FACE_OUTER_BOUND('',#14116,.T.);
#7963=FACE_OUTER_BOUND('',#14117,.T.);
#7964=FACE_OUTER_BOUND('',#14118,.T.);
#7965=FACE_OUTER_BOUND('',#14119,.T.);
#7966=FACE_OUTER_BOUND('',#14120,.T.);
#7967=FACE_OUTER_BOUND('',#14121,.T.);
#7968=FACE_OUTER_BOUND('',#14122,.T.);
#7969=FACE_OUTER_BOUND('',#14123,.T.);
#7970=FACE_OUTER_BOUND('',#14124,.T.);
#7971=FACE_OUTER_BOUND('',#14125,.T.);
#7972=FACE_OUTER_BOUND('',#14126,.T.);
#7973=FACE_OUTER_BOUND('',#14127,.T.);
#7974=FACE_OUTER_BOUND('',#14128,.T.);
#7975=FACE_OUTER_BOUND('',#14129,.T.);
#7976=FACE_OUTER_BOUND('',#14130,.T.);
#7977=FACE_OUTER_BOUND('',#14131,.T.);
#7978=FACE_OUTER_BOUND('',#14132,.T.);
#7979=FACE_OUTER_BOUND('',#14133,.T.);
#7980=FACE_OUTER_BOUND('',#14134,.T.);
#7981=FACE_OUTER_BOUND('',#14135,.T.);
#7982=FACE_OUTER_BOUND('',#14136,.T.);
#7983=FACE_OUTER_BOUND('',#14137,.T.);
#7984=FACE_OUTER_BOUND('',#14138,.T.);
#7985=FACE_OUTER_BOUND('',#14139,.T.);
#7986=FACE_OUTER_BOUND('',#14140,.T.);
#7987=FACE_OUTER_BOUND('',#14141,.T.);
#7988=FACE_OUTER_BOUND('',#14142,.T.);
#7989=FACE_OUTER_BOUND('',#14143,.T.);
#7990=FACE_OUTER_BOUND('',#14144,.T.);
#7991=FACE_OUTER_BOUND('',#14145,.T.);
#7992=FACE_OUTER_BOUND('',#14146,.T.);
#7993=FACE_OUTER_BOUND('',#14147,.T.);
#7994=FACE_OUTER_BOUND('',#14148,.T.);
#7995=FACE_OUTER_BOUND('',#14149,.T.);
#7996=FACE_OUTER_BOUND('',#14150,.T.);
#7997=FACE_OUTER_BOUND('',#14151,.T.);
#7998=FACE_OUTER_BOUND('',#14152,.T.);
#7999=FACE_OUTER_BOUND('',#14153,.T.);
#8000=FACE_OUTER_BOUND('',#14154,.T.);
#8001=FACE_OUTER_BOUND('',#14155,.T.);
#8002=FACE_OUTER_BOUND('',#14156,.T.);
#8003=FACE_OUTER_BOUND('',#14157,.T.);
#8004=FACE_OUTER_BOUND('',#14158,.T.);
#8005=FACE_OUTER_BOUND('',#14159,.T.);
#8006=FACE_OUTER_BOUND('',#14160,.T.);
#8007=FACE_OUTER_BOUND('',#14161,.T.);
#8008=FACE_OUTER_BOUND('',#14162,.T.);
#8009=FACE_OUTER_BOUND('',#14163,.T.);
#8010=FACE_OUTER_BOUND('',#14164,.T.);
#8011=FACE_OUTER_BOUND('',#14165,.T.);
#8012=FACE_OUTER_BOUND('',#14166,.T.);
#8013=FACE_OUTER_BOUND('',#14167,.T.);
#8014=FACE_OUTER_BOUND('',#14168,.T.);
#8015=FACE_OUTER_BOUND('',#14169,.T.);
#8016=FACE_OUTER_BOUND('',#14170,.T.);
#8017=FACE_OUTER_BOUND('',#14171,.T.);
#8018=FACE_OUTER_BOUND('',#14172,.T.);
#8019=FACE_OUTER_BOUND('',#14173,.T.);
#8020=FACE_OUTER_BOUND('',#14174,.T.);
#8021=FACE_OUTER_BOUND('',#14175,.T.);
#8022=FACE_OUTER_BOUND('',#14176,.T.);
#8023=FACE_OUTER_BOUND('',#14177,.T.);
#8024=FACE_OUTER_BOUND('',#14178,.T.);
#8025=FACE_OUTER_BOUND('',#14179,.T.);
#8026=FACE_OUTER_BOUND('',#14180,.T.);
#8027=FACE_OUTER_BOUND('',#14181,.T.);
#8028=FACE_OUTER_BOUND('',#14182,.T.);
#8029=FACE_OUTER_BOUND('',#14183,.T.);
#8030=FACE_OUTER_BOUND('',#14184,.T.);
#8031=FACE_OUTER_BOUND('',#14185,.T.);
#8032=FACE_OUTER_BOUND('',#14186,.T.);
#8033=FACE_OUTER_BOUND('',#14187,.T.);
#8034=FACE_OUTER_BOUND('',#14188,.T.);
#8035=FACE_OUTER_BOUND('',#14189,.T.);
#8036=FACE_OUTER_BOUND('',#14190,.T.);
#8037=FACE_OUTER_BOUND('',#14191,.T.);
#8038=FACE_OUTER_BOUND('',#14192,.T.);
#8039=FACE_OUTER_BOUND('',#14193,.T.);
#8040=FACE_OUTER_BOUND('',#14194,.T.);
#8041=FACE_OUTER_BOUND('',#14195,.T.);
#8042=FACE_OUTER_BOUND('',#14196,.T.);
#8043=FACE_OUTER_BOUND('',#14197,.T.);
#8044=FACE_OUTER_BOUND('',#14198,.T.);
#8045=FACE_OUTER_BOUND('',#14199,.T.);
#8046=FACE_OUTER_BOUND('',#14200,.T.);
#8047=FACE_OUTER_BOUND('',#14201,.T.);
#8048=FACE_OUTER_BOUND('',#14202,.T.);
#8049=FACE_OUTER_BOUND('',#14203,.T.);
#8050=FACE_OUTER_BOUND('',#14204,.T.);
#8051=FACE_OUTER_BOUND('',#14205,.T.);
#8052=FACE_OUTER_BOUND('',#14206,.T.);
#8053=FACE_OUTER_BOUND('',#14207,.T.);
#8054=FACE_OUTER_BOUND('',#14208,.T.);
#8055=FACE_OUTER_BOUND('',#14209,.T.);
#8056=FACE_OUTER_BOUND('',#14210,.T.);
#8057=FACE_OUTER_BOUND('',#14211,.T.);
#8058=FACE_OUTER_BOUND('',#14212,.T.);
#8059=FACE_OUTER_BOUND('',#14213,.T.);
#8060=FACE_OUTER_BOUND('',#14214,.T.);
#8061=FACE_OUTER_BOUND('',#14215,.T.);
#8062=FACE_OUTER_BOUND('',#14216,.T.);
#8063=FACE_OUTER_BOUND('',#14217,.T.);
#8064=FACE_OUTER_BOUND('',#14218,.T.);
#8065=FACE_OUTER_BOUND('',#14219,.T.);
#8066=FACE_OUTER_BOUND('',#14220,.T.);
#8067=FACE_OUTER_BOUND('',#14221,.T.);
#8068=FACE_OUTER_BOUND('',#14222,.T.);
#8069=FACE_OUTER_BOUND('',#14223,.T.);
#8070=FACE_OUTER_BOUND('',#14224,.T.);
#8071=FACE_OUTER_BOUND('',#14225,.T.);
#8072=FACE_OUTER_BOUND('',#14226,.T.);
#8073=FACE_OUTER_BOUND('',#14227,.T.);
#8074=FACE_OUTER_BOUND('',#14228,.T.);
#8075=FACE_OUTER_BOUND('',#14229,.T.);
#8076=FACE_OUTER_BOUND('',#14230,.T.);
#8077=FACE_OUTER_BOUND('',#14231,.T.);
#8078=FACE_OUTER_BOUND('',#14232,.T.);
#8079=FACE_OUTER_BOUND('',#14233,.T.);
#8080=FACE_OUTER_BOUND('',#14234,.T.);
#8081=FACE_OUTER_BOUND('',#14235,.T.);
#8082=FACE_OUTER_BOUND('',#14236,.T.);
#8083=FACE_OUTER_BOUND('',#14237,.T.);
#8084=FACE_OUTER_BOUND('',#14238,.T.);
#8085=FACE_OUTER_BOUND('',#14239,.T.);
#8086=FACE_OUTER_BOUND('',#14240,.T.);
#8087=FACE_OUTER_BOUND('',#14241,.T.);
#8088=FACE_OUTER_BOUND('',#14242,.T.);
#8089=FACE_OUTER_BOUND('',#14243,.T.);
#8090=FACE_OUTER_BOUND('',#14244,.T.);
#8091=FACE_OUTER_BOUND('',#14245,.T.);
#8092=FACE_OUTER_BOUND('',#14246,.T.);
#8093=FACE_OUTER_BOUND('',#14247,.T.);
#8094=FACE_OUTER_BOUND('',#14248,.T.);
#8095=FACE_OUTER_BOUND('',#14249,.T.);
#8096=FACE_OUTER_BOUND('',#14250,.T.);
#8097=FACE_OUTER_BOUND('',#14251,.T.);
#8098=FACE_OUTER_BOUND('',#14252,.T.);
#8099=FACE_OUTER_BOUND('',#14253,.T.);
#8100=FACE_OUTER_BOUND('',#14254,.T.);
#8101=FACE_OUTER_BOUND('',#14255,.T.);
#8102=FACE_OUTER_BOUND('',#14256,.T.);
#8103=FACE_OUTER_BOUND('',#14257,.T.);
#8104=FACE_OUTER_BOUND('',#14258,.T.);
#8105=FACE_OUTER_BOUND('',#14259,.T.);
#8106=FACE_OUTER_BOUND('',#14260,.T.);
#8107=FACE_OUTER_BOUND('',#14261,.T.);
#8108=FACE_OUTER_BOUND('',#14262,.T.);
#8109=FACE_OUTER_BOUND('',#14263,.T.);
#8110=FACE_OUTER_BOUND('',#14264,.T.);
#8111=FACE_OUTER_BOUND('',#14265,.T.);
#8112=FACE_OUTER_BOUND('',#14266,.T.);
#8113=FACE_OUTER_BOUND('',#14267,.T.);
#8114=FACE_OUTER_BOUND('',#14268,.T.);
#8115=FACE_OUTER_BOUND('',#14269,.T.);
#8116=FACE_OUTER_BOUND('',#14270,.T.);
#8117=FACE_OUTER_BOUND('',#14271,.T.);
#8118=FACE_OUTER_BOUND('',#14272,.T.);
#8119=FACE_OUTER_BOUND('',#14273,.T.);
#8120=FACE_OUTER_BOUND('',#14274,.T.);
#8121=FACE_OUTER_BOUND('',#14275,.T.);
#8122=FACE_OUTER_BOUND('',#14276,.T.);
#8123=FACE_OUTER_BOUND('',#14277,.T.);
#8124=FACE_OUTER_BOUND('',#14278,.T.);
#8125=FACE_OUTER_BOUND('',#14279,.T.);
#8126=FACE_OUTER_BOUND('',#14280,.T.);
#8127=FACE_OUTER_BOUND('',#14281,.T.);
#8128=FACE_OUTER_BOUND('',#14282,.T.);
#8129=FACE_OUTER_BOUND('',#14283,.T.);
#8130=FACE_OUTER_BOUND('',#14284,.T.);
#8131=FACE_OUTER_BOUND('',#14285,.T.);
#8132=FACE_OUTER_BOUND('',#14286,.T.);
#8133=FACE_OUTER_BOUND('',#14287,.T.);
#8134=FACE_OUTER_BOUND('',#14288,.T.);
#8135=FACE_OUTER_BOUND('',#14289,.T.);
#8136=FACE_OUTER_BOUND('',#14290,.T.);
#8137=FACE_OUTER_BOUND('',#14291,.T.);
#8138=FACE_OUTER_BOUND('',#14292,.T.);
#8139=FACE_OUTER_BOUND('',#14293,.T.);
#8140=FACE_OUTER_BOUND('',#14294,.T.);
#8141=FACE_OUTER_BOUND('',#14295,.T.);
#8142=FACE_OUTER_BOUND('',#14296,.T.);
#8143=FACE_OUTER_BOUND('',#14297,.T.);
#8144=FACE_OUTER_BOUND('',#14298,.T.);
#8145=FACE_OUTER_BOUND('',#14299,.T.);
#8146=FACE_OUTER_BOUND('',#14300,.T.);
#8147=FACE_OUTER_BOUND('',#14301,.T.);
#8148=FACE_OUTER_BOUND('',#14302,.T.);
#8149=FACE_OUTER_BOUND('',#14303,.T.);
#8150=FACE_OUTER_BOUND('',#14304,.T.);
#8151=FACE_OUTER_BOUND('',#14305,.T.);
#8152=FACE_OUTER_BOUND('',#14306,.T.);
#8153=FACE_OUTER_BOUND('',#14307,.T.);
#8154=FACE_OUTER_BOUND('',#14308,.T.);
#8155=FACE_OUTER_BOUND('',#14309,.T.);
#8156=FACE_OUTER_BOUND('',#14310,.T.);
#8157=FACE_OUTER_BOUND('',#14311,.T.);
#8158=FACE_OUTER_BOUND('',#14312,.T.);
#8159=FACE_OUTER_BOUND('',#14313,.T.);
#8160=FACE_OUTER_BOUND('',#14314,.T.);
#8161=FACE_OUTER_BOUND('',#14315,.T.);
#8162=FACE_OUTER_BOUND('',#14316,.T.);
#8163=FACE_OUTER_BOUND('',#14317,.T.);
#8164=FACE_OUTER_BOUND('',#14318,.T.);
#8165=FACE_OUTER_BOUND('',#14319,.T.);
#8166=FACE_OUTER_BOUND('',#14320,.T.);
#8167=FACE_OUTER_BOUND('',#14321,.T.);
#8168=FACE_OUTER_BOUND('',#14322,.T.);
#8169=FACE_OUTER_BOUND('',#14323,.T.);
#8170=FACE_OUTER_BOUND('',#14324,.T.);
#8171=FACE_OUTER_BOUND('',#14325,.T.);
#8172=FACE_OUTER_BOUND('',#14326,.T.);
#8173=FACE_OUTER_BOUND('',#14327,.T.);
#8174=FACE_OUTER_BOUND('',#14328,.T.);
#8175=FACE_OUTER_BOUND('',#14329,.T.);
#8176=FACE_OUTER_BOUND('',#14330,.T.);
#8177=FACE_OUTER_BOUND('',#14331,.T.);
#8178=FACE_OUTER_BOUND('',#14332,.T.);
#8179=FACE_OUTER_BOUND('',#14333,.T.);
#8180=FACE_OUTER_BOUND('',#14334,.T.);
#8181=FACE_OUTER_BOUND('',#14335,.T.);
#8182=FACE_OUTER_BOUND('',#14336,.T.);
#8183=FACE_OUTER_BOUND('',#14337,.T.);
#8184=FACE_OUTER_BOUND('',#14338,.T.);
#8185=FACE_OUTER_BOUND('',#14339,.T.);
#8186=FACE_OUTER_BOUND('',#14340,.T.);
#8187=FACE_OUTER_BOUND('',#14341,.T.);
#8188=FACE_OUTER_BOUND('',#14342,.T.);
#8189=FACE_OUTER_BOUND('',#14343,.T.);
#8190=FACE_OUTER_BOUND('',#14344,.T.);
#8191=FACE_OUTER_BOUND('',#14345,.T.);
#8192=FACE_OUTER_BOUND('',#14346,.T.);
#8193=FACE_OUTER_BOUND('',#14347,.T.);
#8194=FACE_OUTER_BOUND('',#14348,.T.);
#8195=FACE_OUTER_BOUND('',#14349,.T.);
#8196=FACE_OUTER_BOUND('',#14350,.T.);
#8197=FACE_OUTER_BOUND('',#14351,.T.);
#8198=FACE_OUTER_BOUND('',#14352,.T.);
#8199=FACE_OUTER_BOUND('',#14353,.T.);
#8200=FACE_OUTER_BOUND('',#14354,.T.);
#8201=FACE_OUTER_BOUND('',#14355,.T.);
#8202=FACE_OUTER_BOUND('',#14356,.T.);
#8203=FACE_OUTER_BOUND('',#14357,.T.);
#8204=FACE_OUTER_BOUND('',#14358,.T.);
#8205=FACE_OUTER_BOUND('',#14359,.T.);
#8206=FACE_OUTER_BOUND('',#14360,.T.);
#8207=FACE_OUTER_BOUND('',#14361,.T.);
#8208=FACE_OUTER_BOUND('',#14362,.T.);
#8209=FACE_OUTER_BOUND('',#14363,.T.);
#8210=FACE_OUTER_BOUND('',#14364,.T.);
#8211=FACE_OUTER_BOUND('',#14365,.T.);
#8212=FACE_OUTER_BOUND('',#14366,.T.);
#8213=FACE_OUTER_BOUND('',#14367,.T.);
#8214=FACE_OUTER_BOUND('',#14368,.T.);
#8215=FACE_OUTER_BOUND('',#14369,.T.);
#8216=FACE_OUTER_BOUND('',#14370,.T.);
#8217=FACE_OUTER_BOUND('',#14371,.T.);
#8218=FACE_OUTER_BOUND('',#14372,.T.);
#8219=FACE_OUTER_BOUND('',#14373,.T.);
#8220=FACE_OUTER_BOUND('',#14374,.T.);
#8221=FACE_OUTER_BOUND('',#14375,.T.);
#8222=FACE_OUTER_BOUND('',#14376,.T.);
#8223=FACE_OUTER_BOUND('',#14377,.T.);
#8224=FACE_OUTER_BOUND('',#14378,.T.);
#8225=FACE_OUTER_BOUND('',#14379,.T.);
#8226=FACE_OUTER_BOUND('',#14380,.T.);
#8227=FACE_OUTER_BOUND('',#14381,.T.);
#8228=FACE_OUTER_BOUND('',#14382,.T.);
#8229=FACE_OUTER_BOUND('',#14383,.T.);
#8230=FACE_OUTER_BOUND('',#14384,.T.);
#8231=FACE_OUTER_BOUND('',#14385,.T.);
#8232=FACE_OUTER_BOUND('',#14386,.T.);
#8233=FACE_OUTER_BOUND('',#14387,.T.);
#8234=FACE_OUTER_BOUND('',#14388,.T.);
#8235=FACE_OUTER_BOUND('',#14389,.T.);
#8236=FACE_OUTER_BOUND('',#14390,.T.);
#8237=FACE_OUTER_BOUND('',#14391,.T.);
#8238=FACE_OUTER_BOUND('',#14392,.T.);
#8239=FACE_OUTER_BOUND('',#14393,.T.);
#8240=FACE_OUTER_BOUND('',#14394,.T.);
#8241=FACE_OUTER_BOUND('',#14395,.T.);
#8242=FACE_OUTER_BOUND('',#14396,.T.);
#8243=FACE_OUTER_BOUND('',#14397,.T.);
#8244=FACE_OUTER_BOUND('',#14398,.T.);
#8245=FACE_OUTER_BOUND('',#14399,.T.);
#8246=FACE_OUTER_BOUND('',#14400,.T.);
#8247=FACE_OUTER_BOUND('',#14401,.T.);
#8248=FACE_OUTER_BOUND('',#14402,.T.);
#8249=FACE_OUTER_BOUND('',#14403,.T.);
#8250=FACE_OUTER_BOUND('',#14404,.T.);
#8251=FACE_OUTER_BOUND('',#14405,.T.);
#8252=FACE_OUTER_BOUND('',#14406,.T.);
#8253=FACE_OUTER_BOUND('',#14407,.T.);
#8254=FACE_OUTER_BOUND('',#14408,.T.);
#8255=FACE_OUTER_BOUND('',#14409,.T.);
#8256=FACE_OUTER_BOUND('',#14410,.T.);
#8257=FACE_OUTER_BOUND('',#14411,.T.);
#8258=FACE_OUTER_BOUND('',#14412,.T.);
#8259=FACE_OUTER_BOUND('',#14413,.T.);
#8260=FACE_OUTER_BOUND('',#14414,.T.);
#8261=FACE_OUTER_BOUND('',#14415,.T.);
#8262=FACE_OUTER_BOUND('',#14416,.T.);
#8263=FACE_OUTER_BOUND('',#14417,.T.);
#8264=FACE_OUTER_BOUND('',#14418,.T.);
#8265=FACE_OUTER_BOUND('',#14419,.T.);
#8266=FACE_OUTER_BOUND('',#14420,.T.);
#8267=FACE_OUTER_BOUND('',#14421,.T.);
#8268=FACE_OUTER_BOUND('',#14422,.T.);
#8269=FACE_OUTER_BOUND('',#14423,.T.);
#8270=FACE_OUTER_BOUND('',#14424,.T.);
#8271=FACE_OUTER_BOUND('',#14425,.T.);
#8272=FACE_OUTER_BOUND('',#14426,.T.);
#8273=FACE_OUTER_BOUND('',#14427,.T.);
#8274=FACE_OUTER_BOUND('',#14428,.T.);
#8275=FACE_OUTER_BOUND('',#14429,.T.);
#8276=FACE_OUTER_BOUND('',#14430,.T.);
#8277=FACE_OUTER_BOUND('',#14431,.T.);
#8278=FACE_OUTER_BOUND('',#14432,.T.);
#8279=FACE_OUTER_BOUND('',#14433,.T.);
#8280=FACE_OUTER_BOUND('',#14434,.T.);
#8281=FACE_OUTER_BOUND('',#14435,.T.);
#8282=FACE_OUTER_BOUND('',#14436,.T.);
#8283=FACE_OUTER_BOUND('',#14437,.T.);
#8284=FACE_OUTER_BOUND('',#14438,.T.);
#8285=FACE_OUTER_BOUND('',#14439,.T.);
#8286=FACE_OUTER_BOUND('',#14440,.T.);
#8287=FACE_OUTER_BOUND('',#14441,.T.);
#8288=FACE_OUTER_BOUND('',#14442,.T.);
#8289=FACE_OUTER_BOUND('',#14443,.T.);
#8290=FACE_OUTER_BOUND('',#14444,.T.);
#8291=FACE_OUTER_BOUND('',#14445,.T.);
#8292=FACE_OUTER_BOUND('',#14446,.T.);
#8293=FACE_OUTER_BOUND('',#14447,.T.);
#8294=FACE_OUTER_BOUND('',#14448,.T.);
#8295=FACE_OUTER_BOUND('',#14449,.T.);
#8296=FACE_OUTER_BOUND('',#14450,.T.);
#8297=FACE_OUTER_BOUND('',#14451,.T.);
#8298=FACE_OUTER_BOUND('',#14452,.T.);
#8299=FACE_OUTER_BOUND('',#14453,.T.);
#8300=FACE_OUTER_BOUND('',#14454,.T.);
#8301=FACE_OUTER_BOUND('',#14455,.T.);
#8302=FACE_OUTER_BOUND('',#14456,.T.);
#8303=FACE_OUTER_BOUND('',#14457,.T.);
#8304=FACE_OUTER_BOUND('',#14458,.T.);
#8305=FACE_OUTER_BOUND('',#14459,.T.);
#8306=FACE_OUTER_BOUND('',#14460,.T.);
#8307=FACE_OUTER_BOUND('',#14461,.T.);
#8308=FACE_OUTER_BOUND('',#14462,.T.);
#8309=FACE_OUTER_BOUND('',#14463,.T.);
#8310=FACE_OUTER_BOUND('',#14464,.T.);
#8311=FACE_OUTER_BOUND('',#14465,.T.);
#8312=FACE_OUTER_BOUND('',#14466,.T.);
#8313=FACE_OUTER_BOUND('',#14467,.T.);
#8314=FACE_OUTER_BOUND('',#14468,.T.);
#8315=FACE_OUTER_BOUND('',#14469,.T.);
#8316=FACE_OUTER_BOUND('',#14470,.T.);
#8317=FACE_OUTER_BOUND('',#14471,.T.);
#8318=FACE_OUTER_BOUND('',#14472,.T.);
#8319=FACE_OUTER_BOUND('',#14473,.T.);
#8320=FACE_OUTER_BOUND('',#14474,.T.);
#8321=FACE_OUTER_BOUND('',#14476,.T.);
#8322=FACE_OUTER_BOUND('',#14477,.T.);
#8323=FACE_OUTER_BOUND('',#14478,.T.);
#8324=FACE_OUTER_BOUND('',#14479,.T.);
#8325=FACE_OUTER_BOUND('',#14480,.T.);
#8326=FACE_OUTER_BOUND('',#14481,.T.);
#8327=FACE_OUTER_BOUND('',#14483,.T.);
#8328=FACE_OUTER_BOUND('',#14485,.T.);
#8329=FACE_OUTER_BOUND('',#14486,.T.);
#8330=FACE_OUTER_BOUND('',#14487,.T.);
#8331=FACE_OUTER_BOUND('',#14488,.T.);
#8332=FACE_OUTER_BOUND('',#14489,.T.);
#8333=FACE_OUTER_BOUND('',#14490,.T.);
#8334=FACE_OUTER_BOUND('',#14491,.T.);
#8335=FACE_OUTER_BOUND('',#14492,.T.);
#8336=FACE_OUTER_BOUND('',#14493,.T.);
#8337=FACE_OUTER_BOUND('',#14494,.T.);
#8338=FACE_OUTER_BOUND('',#14495,.T.);
#8339=FACE_OUTER_BOUND('',#14496,.T.);
#8340=FACE_OUTER_BOUND('',#14497,.T.);
#8341=FACE_OUTER_BOUND('',#14498,.T.);
#8342=FACE_OUTER_BOUND('',#14499,.T.);
#8343=FACE_OUTER_BOUND('',#14500,.T.);
#8344=FACE_OUTER_BOUND('',#14501,.T.);
#8345=FACE_OUTER_BOUND('',#14502,.T.);
#8346=FACE_OUTER_BOUND('',#14503,.T.);
#8347=FACE_OUTER_BOUND('',#14504,.T.);
#8348=FACE_OUTER_BOUND('',#14505,.T.);
#8349=FACE_OUTER_BOUND('',#14506,.T.);
#8350=FACE_OUTER_BOUND('',#14507,.T.);
#8351=FACE_OUTER_BOUND('',#14508,.T.);
#8352=FACE_OUTER_BOUND('',#14509,.T.);
#8353=FACE_OUTER_BOUND('',#14510,.T.);
#8354=FACE_OUTER_BOUND('',#14511,.T.);
#8355=FACE_OUTER_BOUND('',#14512,.T.);
#8356=FACE_OUTER_BOUND('',#14513,.T.);
#8357=FACE_OUTER_BOUND('',#14514,.T.);
#8358=FACE_OUTER_BOUND('',#14515,.T.);
#8359=FACE_OUTER_BOUND('',#14516,.T.);
#8360=FACE_OUTER_BOUND('',#14517,.T.);
#8361=FACE_OUTER_BOUND('',#14518,.T.);
#8362=FACE_OUTER_BOUND('',#14519,.T.);
#8363=FACE_OUTER_BOUND('',#14520,.T.);
#8364=FACE_OUTER_BOUND('',#14521,.T.);
#8365=FACE_OUTER_BOUND('',#14522,.T.);
#8366=FACE_OUTER_BOUND('',#14523,.T.);
#8367=FACE_OUTER_BOUND('',#14524,.T.);
#8368=FACE_OUTER_BOUND('',#14525,.T.);
#8369=FACE_OUTER_BOUND('',#14526,.T.);
#8370=FACE_OUTER_BOUND('',#14527,.T.);
#8371=FACE_OUTER_BOUND('',#14528,.T.);
#8372=FACE_OUTER_BOUND('',#14529,.T.);
#8373=FACE_OUTER_BOUND('',#14530,.T.);
#8374=FACE_OUTER_BOUND('',#14531,.T.);
#8375=FACE_OUTER_BOUND('',#14532,.T.);
#8376=FACE_OUTER_BOUND('',#14533,.T.);
#8377=FACE_OUTER_BOUND('',#14534,.T.);
#8378=FACE_OUTER_BOUND('',#14535,.T.);
#8379=FACE_OUTER_BOUND('',#14536,.T.);
#8380=FACE_OUTER_BOUND('',#14537,.T.);
#8381=FACE_OUTER_BOUND('',#14538,.T.);
#8382=FACE_OUTER_BOUND('',#14539,.T.);
#8383=FACE_OUTER_BOUND('',#14540,.T.);
#8384=FACE_OUTER_BOUND('',#14541,.T.);
#8385=FACE_OUTER_BOUND('',#14542,.T.);
#8386=FACE_OUTER_BOUND('',#14543,.T.);
#8387=FACE_OUTER_BOUND('',#14544,.T.);
#8388=FACE_OUTER_BOUND('',#14545,.T.);
#8389=FACE_OUTER_BOUND('',#14546,.T.);
#8390=FACE_OUTER_BOUND('',#14547,.T.);
#8391=FACE_OUTER_BOUND('',#14548,.T.);
#8392=FACE_OUTER_BOUND('',#14549,.T.);
#8393=FACE_OUTER_BOUND('',#14550,.T.);
#8394=FACE_OUTER_BOUND('',#14551,.T.);
#8395=FACE_OUTER_BOUND('',#14552,.T.);
#8396=FACE_OUTER_BOUND('',#14553,.T.);
#8397=FACE_OUTER_BOUND('',#14554,.T.);
#8398=FACE_OUTER_BOUND('',#14555,.T.);
#8399=FACE_OUTER_BOUND('',#14556,.T.);
#8400=FACE_OUTER_BOUND('',#14557,.T.);
#8401=FACE_OUTER_BOUND('',#14558,.T.);
#8402=FACE_OUTER_BOUND('',#14559,.T.);
#8403=FACE_OUTER_BOUND('',#14560,.T.);
#8404=FACE_OUTER_BOUND('',#14561,.T.);
#8405=FACE_OUTER_BOUND('',#14562,.T.);
#8406=FACE_OUTER_BOUND('',#14563,.T.);
#8407=FACE_OUTER_BOUND('',#14564,.T.);
#8408=FACE_OUTER_BOUND('',#14565,.T.);
#8409=FACE_OUTER_BOUND('',#14566,.T.);
#8410=FACE_OUTER_BOUND('',#14567,.T.);
#8411=FACE_OUTER_BOUND('',#14568,.T.);
#8412=FACE_OUTER_BOUND('',#14569,.T.);
#8413=FACE_OUTER_BOUND('',#14570,.T.);
#8414=FACE_OUTER_BOUND('',#14571,.T.);
#8415=FACE_OUTER_BOUND('',#14572,.T.);
#8416=FACE_OUTER_BOUND('',#14573,.T.);
#8417=FACE_OUTER_BOUND('',#14574,.T.);
#8418=FACE_OUTER_BOUND('',#14575,.T.);
#8419=FACE_OUTER_BOUND('',#14576,.T.);
#8420=FACE_OUTER_BOUND('',#14577,.T.);
#8421=FACE_OUTER_BOUND('',#14578,.T.);
#8422=FACE_OUTER_BOUND('',#14579,.T.);
#8423=FACE_OUTER_BOUND('',#14580,.T.);
#8424=FACE_OUTER_BOUND('',#14581,.T.);
#8425=FACE_OUTER_BOUND('',#14582,.T.);
#8426=FACE_OUTER_BOUND('',#14583,.T.);
#8427=FACE_OUTER_BOUND('',#14584,.T.);
#8428=FACE_OUTER_BOUND('',#14585,.T.);
#8429=FACE_OUTER_BOUND('',#14586,.T.);
#8430=FACE_OUTER_BOUND('',#14587,.T.);
#8431=FACE_OUTER_BOUND('',#14588,.T.);
#8432=FACE_OUTER_BOUND('',#14589,.T.);
#8433=FACE_OUTER_BOUND('',#14590,.T.);
#8434=FACE_OUTER_BOUND('',#14591,.T.);
#8435=FACE_OUTER_BOUND('',#14592,.T.);
#8436=FACE_OUTER_BOUND('',#14593,.T.);
#8437=FACE_OUTER_BOUND('',#14594,.T.);
#8438=FACE_OUTER_BOUND('',#14595,.T.);
#8439=FACE_OUTER_BOUND('',#14596,.T.);
#8440=FACE_OUTER_BOUND('',#14597,.T.);
#8441=FACE_OUTER_BOUND('',#14598,.T.);
#8442=FACE_OUTER_BOUND('',#14599,.T.);
#8443=FACE_OUTER_BOUND('',#14600,.T.);
#8444=FACE_OUTER_BOUND('',#14601,.T.);
#8445=FACE_OUTER_BOUND('',#14602,.T.);
#8446=FACE_OUTER_BOUND('',#14603,.T.);
#8447=FACE_OUTER_BOUND('',#14604,.T.);
#8448=FACE_OUTER_BOUND('',#14605,.T.);
#8449=FACE_OUTER_BOUND('',#14606,.T.);
#8450=FACE_OUTER_BOUND('',#14607,.T.);
#8451=FACE_OUTER_BOUND('',#14608,.T.);
#8452=FACE_OUTER_BOUND('',#14609,.T.);
#8453=FACE_OUTER_BOUND('',#14610,.T.);
#8454=FACE_OUTER_BOUND('',#14611,.T.);
#8455=FACE_OUTER_BOUND('',#14612,.T.);
#8456=FACE_OUTER_BOUND('',#14613,.T.);
#8457=FACE_OUTER_BOUND('',#14614,.T.);
#8458=FACE_OUTER_BOUND('',#14615,.T.);
#8459=FACE_OUTER_BOUND('',#14616,.T.);
#8460=FACE_OUTER_BOUND('',#14617,.T.);
#8461=FACE_OUTER_BOUND('',#14618,.T.);
#8462=FACE_OUTER_BOUND('',#14619,.T.);
#8463=FACE_OUTER_BOUND('',#14620,.T.);
#8464=FACE_OUTER_BOUND('',#14621,.T.);
#8465=FACE_OUTER_BOUND('',#14622,.T.);
#8466=FACE_OUTER_BOUND('',#14623,.T.);
#8467=FACE_OUTER_BOUND('',#14624,.T.);
#8468=FACE_OUTER_BOUND('',#14625,.T.);
#8469=FACE_OUTER_BOUND('',#14626,.T.);
#8470=FACE_OUTER_BOUND('',#14627,.T.);
#8471=FACE_OUTER_BOUND('',#14628,.T.);
#8472=FACE_OUTER_BOUND('',#14629,.T.);
#8473=FACE_OUTER_BOUND('',#14630,.T.);
#8474=FACE_OUTER_BOUND('',#14631,.T.);
#8475=FACE_OUTER_BOUND('',#14632,.T.);
#8476=FACE_OUTER_BOUND('',#14633,.T.);
#8477=FACE_OUTER_BOUND('',#14634,.T.);
#8478=FACE_OUTER_BOUND('',#14635,.T.);
#8479=FACE_OUTER_BOUND('',#14636,.T.);
#8480=FACE_OUTER_BOUND('',#14637,.T.);
#8481=FACE_OUTER_BOUND('',#14638,.T.);
#8482=FACE_OUTER_BOUND('',#14639,.T.);
#8483=FACE_OUTER_BOUND('',#14640,.T.);
#8484=FACE_OUTER_BOUND('',#14641,.T.);
#8485=FACE_OUTER_BOUND('',#14642,.T.);
#8486=FACE_OUTER_BOUND('',#14643,.T.);
#8487=FACE_OUTER_BOUND('',#14644,.T.);
#8488=FACE_OUTER_BOUND('',#14645,.T.);
#8489=FACE_OUTER_BOUND('',#14646,.T.);
#8490=FACE_OUTER_BOUND('',#14647,.T.);
#8491=FACE_OUTER_BOUND('',#14648,.T.);
#8492=FACE_OUTER_BOUND('',#14649,.T.);
#8493=FACE_OUTER_BOUND('',#14650,.T.);
#8494=FACE_OUTER_BOUND('',#14651,.T.);
#8495=FACE_OUTER_BOUND('',#14652,.T.);
#8496=FACE_OUTER_BOUND('',#14653,.T.);
#8497=FACE_OUTER_BOUND('',#14654,.T.);
#8498=FACE_OUTER_BOUND('',#14655,.T.);
#8499=FACE_OUTER_BOUND('',#14656,.T.);
#8500=FACE_OUTER_BOUND('',#14657,.T.);
#8501=FACE_OUTER_BOUND('',#14658,.T.);
#8502=FACE_OUTER_BOUND('',#14659,.T.);
#8503=FACE_OUTER_BOUND('',#14660,.T.);
#8504=FACE_OUTER_BOUND('',#14661,.T.);
#8505=FACE_OUTER_BOUND('',#14662,.T.);
#8506=FACE_OUTER_BOUND('',#14663,.T.);
#8507=FACE_OUTER_BOUND('',#14664,.T.);
#8508=FACE_OUTER_BOUND('',#14665,.T.);
#8509=FACE_OUTER_BOUND('',#14666,.T.);
#8510=FACE_OUTER_BOUND('',#14667,.T.);
#8511=FACE_OUTER_BOUND('',#14668,.T.);
#8512=FACE_OUTER_BOUND('',#14669,.T.);
#8513=FACE_OUTER_BOUND('',#14670,.T.);
#8514=FACE_OUTER_BOUND('',#14671,.T.);
#8515=FACE_OUTER_BOUND('',#14672,.T.);
#8516=FACE_OUTER_BOUND('',#14673,.T.);
#8517=FACE_OUTER_BOUND('',#14674,.T.);
#8518=FACE_OUTER_BOUND('',#14675,.T.);
#8519=FACE_OUTER_BOUND('',#14676,.T.);
#8520=FACE_OUTER_BOUND('',#14677,.T.);
#8521=FACE_OUTER_BOUND('',#14678,.T.);
#8522=FACE_OUTER_BOUND('',#14679,.T.);
#8523=FACE_OUTER_BOUND('',#14680,.T.);
#8524=FACE_OUTER_BOUND('',#14681,.T.);
#8525=FACE_OUTER_BOUND('',#14682,.T.);
#8526=FACE_OUTER_BOUND('',#14683,.T.);
#8527=FACE_OUTER_BOUND('',#14684,.T.);
#8528=FACE_OUTER_BOUND('',#14685,.T.);
#8529=FACE_OUTER_BOUND('',#14686,.T.);
#8530=FACE_OUTER_BOUND('',#14687,.T.);
#8531=FACE_OUTER_BOUND('',#14688,.T.);
#8532=FACE_OUTER_BOUND('',#14689,.T.);
#8533=FACE_OUTER_BOUND('',#14690,.T.);
#8534=FACE_OUTER_BOUND('',#14691,.T.);
#8535=FACE_OUTER_BOUND('',#14692,.T.);
#8536=FACE_OUTER_BOUND('',#14693,.T.);
#8537=FACE_OUTER_BOUND('',#14694,.T.);
#8538=FACE_OUTER_BOUND('',#14695,.T.);
#8539=FACE_OUTER_BOUND('',#14696,.T.);
#8540=FACE_OUTER_BOUND('',#14697,.T.);
#8541=FACE_OUTER_BOUND('',#14698,.T.);
#8542=FACE_OUTER_BOUND('',#14699,.T.);
#8543=FACE_OUTER_BOUND('',#14700,.T.);
#8544=FACE_OUTER_BOUND('',#14701,.T.);
#8545=FACE_OUTER_BOUND('',#14702,.T.);
#8546=FACE_OUTER_BOUND('',#14703,.T.);
#8547=FACE_OUTER_BOUND('',#14704,.T.);
#8548=FACE_OUTER_BOUND('',#14705,.T.);
#8549=FACE_OUTER_BOUND('',#14706,.T.);
#8550=FACE_OUTER_BOUND('',#14707,.T.);
#8551=FACE_OUTER_BOUND('',#14708,.T.);
#8552=FACE_OUTER_BOUND('',#14709,.T.);
#8553=FACE_OUTER_BOUND('',#14710,.T.);
#8554=FACE_OUTER_BOUND('',#14711,.T.);
#8555=FACE_OUTER_BOUND('',#14712,.T.);
#8556=FACE_OUTER_BOUND('',#14713,.T.);
#8557=FACE_OUTER_BOUND('',#14714,.T.);
#8558=FACE_OUTER_BOUND('',#14715,.T.);
#8559=FACE_OUTER_BOUND('',#14716,.T.);
#8560=FACE_OUTER_BOUND('',#14717,.T.);
#8561=FACE_OUTER_BOUND('',#14718,.T.);
#8562=FACE_OUTER_BOUND('',#14719,.T.);
#8563=FACE_OUTER_BOUND('',#14720,.T.);
#8564=FACE_OUTER_BOUND('',#14721,.T.);
#8565=FACE_OUTER_BOUND('',#14722,.T.);
#8566=FACE_OUTER_BOUND('',#14723,.T.);
#8567=FACE_OUTER_BOUND('',#14724,.T.);
#8568=FACE_OUTER_BOUND('',#14725,.T.);
#8569=FACE_OUTER_BOUND('',#14726,.T.);
#8570=FACE_OUTER_BOUND('',#14727,.T.);
#8571=FACE_OUTER_BOUND('',#14728,.T.);
#8572=FACE_OUTER_BOUND('',#14729,.T.);
#8573=FACE_OUTER_BOUND('',#14730,.T.);
#8574=FACE_OUTER_BOUND('',#14731,.T.);
#8575=FACE_OUTER_BOUND('',#14732,.T.);
#8576=FACE_OUTER_BOUND('',#14733,.T.);
#8577=FACE_OUTER_BOUND('',#14734,.T.);
#8578=FACE_OUTER_BOUND('',#14735,.T.);
#8579=FACE_OUTER_BOUND('',#14736,.T.);
#8580=FACE_OUTER_BOUND('',#14737,.T.);
#8581=FACE_OUTER_BOUND('',#14738,.T.);
#8582=FACE_OUTER_BOUND('',#14739,.T.);
#8583=FACE_OUTER_BOUND('',#14740,.T.);
#8584=FACE_OUTER_BOUND('',#14741,.T.);
#8585=FACE_OUTER_BOUND('',#14742,.T.);
#8586=FACE_OUTER_BOUND('',#14743,.T.);
#8587=FACE_OUTER_BOUND('',#14744,.T.);
#8588=FACE_OUTER_BOUND('',#14745,.T.);
#8589=FACE_OUTER_BOUND('',#14746,.T.);
#8590=FACE_OUTER_BOUND('',#14747,.T.);
#8591=FACE_OUTER_BOUND('',#14748,.T.);
#8592=FACE_OUTER_BOUND('',#14749,.T.);
#8593=FACE_OUTER_BOUND('',#14750,.T.);
#8594=FACE_OUTER_BOUND('',#14751,.T.);
#8595=FACE_OUTER_BOUND('',#14752,.T.);
#8596=FACE_OUTER_BOUND('',#14753,.T.);
#8597=FACE_OUTER_BOUND('',#14754,.T.);
#8598=FACE_OUTER_BOUND('',#14755,.T.);
#8599=FACE_OUTER_BOUND('',#14756,.T.);
#8600=FACE_OUTER_BOUND('',#14757,.T.);
#8601=FACE_OUTER_BOUND('',#14758,.T.);
#8602=FACE_OUTER_BOUND('',#14759,.T.);
#8603=FACE_OUTER_BOUND('',#14760,.T.);
#8604=FACE_OUTER_BOUND('',#14761,.T.);
#8605=FACE_OUTER_BOUND('',#14762,.T.);
#8606=FACE_OUTER_BOUND('',#14763,.T.);
#8607=FACE_OUTER_BOUND('',#14764,.T.);
#8608=FACE_OUTER_BOUND('',#14765,.T.);
#8609=FACE_OUTER_BOUND('',#14766,.T.);
#8610=FACE_OUTER_BOUND('',#14767,.T.);
#8611=FACE_OUTER_BOUND('',#14768,.T.);
#8612=FACE_OUTER_BOUND('',#14769,.T.);
#8613=FACE_OUTER_BOUND('',#14770,.T.);
#8614=FACE_OUTER_BOUND('',#14771,.T.);
#8615=FACE_OUTER_BOUND('',#14772,.T.);
#8616=FACE_OUTER_BOUND('',#14773,.T.);
#8617=FACE_OUTER_BOUND('',#14774,.T.);
#8618=FACE_OUTER_BOUND('',#14775,.T.);
#8619=FACE_OUTER_BOUND('',#14776,.T.);
#8620=FACE_OUTER_BOUND('',#14777,.T.);
#8621=FACE_OUTER_BOUND('',#14778,.T.);
#8622=FACE_OUTER_BOUND('',#14779,.T.);
#8623=FACE_OUTER_BOUND('',#14780,.T.);
#8624=FACE_OUTER_BOUND('',#14781,.T.);
#8625=FACE_OUTER_BOUND('',#14782,.T.);
#8626=FACE_OUTER_BOUND('',#14783,.T.);
#8627=FACE_OUTER_BOUND('',#14784,.T.);
#8628=FACE_OUTER_BOUND('',#14785,.T.);
#8629=FACE_OUTER_BOUND('',#14786,.T.);
#8630=FACE_OUTER_BOUND('',#14787,.T.);
#8631=FACE_OUTER_BOUND('',#14788,.T.);
#8632=FACE_OUTER_BOUND('',#14789,.T.);
#8633=FACE_OUTER_BOUND('',#14790,.T.);
#8634=FACE_OUTER_BOUND('',#14791,.T.);
#8635=FACE_OUTER_BOUND('',#14792,.T.);
#8636=FACE_OUTER_BOUND('',#14793,.T.);
#8637=FACE_OUTER_BOUND('',#14794,.T.);
#8638=FACE_OUTER_BOUND('',#14795,.T.);
#8639=FACE_OUTER_BOUND('',#14796,.T.);
#8640=FACE_OUTER_BOUND('',#14797,.T.);
#8641=FACE_OUTER_BOUND('',#14798,.T.);
#8642=FACE_OUTER_BOUND('',#14799,.T.);
#8643=FACE_OUTER_BOUND('',#14800,.T.);
#8644=FACE_OUTER_BOUND('',#14801,.T.);
#8645=FACE_OUTER_BOUND('',#14802,.T.);
#8646=FACE_OUTER_BOUND('',#14803,.T.);
#8647=FACE_OUTER_BOUND('',#14804,.T.);
#8648=FACE_OUTER_BOUND('',#14805,.T.);
#8649=FACE_OUTER_BOUND('',#14806,.T.);
#8650=FACE_OUTER_BOUND('',#14807,.T.);
#8651=FACE_OUTER_BOUND('',#14808,.T.);
#8652=FACE_OUTER_BOUND('',#14809,.T.);
#8653=FACE_OUTER_BOUND('',#14810,.T.);
#8654=FACE_OUTER_BOUND('',#14811,.T.);
#8655=FACE_OUTER_BOUND('',#14812,.T.);
#8656=FACE_OUTER_BOUND('',#14813,.T.);
#8657=FACE_OUTER_BOUND('',#14814,.T.);
#8658=FACE_OUTER_BOUND('',#14815,.T.);
#8659=FACE_OUTER_BOUND('',#14816,.T.);
#8660=FACE_OUTER_BOUND('',#14817,.T.);
#8661=FACE_OUTER_BOUND('',#14818,.T.);
#8662=FACE_OUTER_BOUND('',#14819,.T.);
#8663=FACE_OUTER_BOUND('',#14820,.T.);
#8664=FACE_OUTER_BOUND('',#14821,.T.);
#8665=FACE_OUTER_BOUND('',#14822,.T.);
#8666=FACE_OUTER_BOUND('',#14823,.T.);
#8667=FACE_OUTER_BOUND('',#14824,.T.);
#8668=FACE_OUTER_BOUND('',#14825,.T.);
#8669=FACE_OUTER_BOUND('',#14826,.T.);
#8670=FACE_OUTER_BOUND('',#14827,.T.);
#8671=FACE_OUTER_BOUND('',#14828,.T.);
#8672=FACE_OUTER_BOUND('',#14829,.T.);
#8673=FACE_OUTER_BOUND('',#14830,.T.);
#8674=FACE_OUTER_BOUND('',#14831,.T.);
#8675=FACE_OUTER_BOUND('',#14832,.T.);
#8676=FACE_OUTER_BOUND('',#14833,.T.);
#8677=FACE_OUTER_BOUND('',#14834,.T.);
#8678=FACE_OUTER_BOUND('',#14835,.T.);
#8679=FACE_OUTER_BOUND('',#14836,.T.);
#8680=FACE_OUTER_BOUND('',#14837,.T.);
#8681=FACE_OUTER_BOUND('',#14838,.T.);
#8682=FACE_OUTER_BOUND('',#14839,.T.);
#8683=FACE_OUTER_BOUND('',#14840,.T.);
#8684=FACE_OUTER_BOUND('',#14841,.T.);
#8685=FACE_OUTER_BOUND('',#14842,.T.);
#8686=FACE_OUTER_BOUND('',#14843,.T.);
#8687=FACE_OUTER_BOUND('',#14844,.T.);
#8688=FACE_OUTER_BOUND('',#14845,.T.);
#8689=FACE_OUTER_BOUND('',#14846,.T.);
#8690=FACE_OUTER_BOUND('',#14847,.T.);
#8691=FACE_OUTER_BOUND('',#14848,.T.);
#8692=FACE_OUTER_BOUND('',#14849,.T.);
#8693=FACE_OUTER_BOUND('',#14850,.T.);
#8694=FACE_OUTER_BOUND('',#14851,.T.);
#8695=FACE_OUTER_BOUND('',#14852,.T.);
#8696=FACE_OUTER_BOUND('',#14853,.T.);
#8697=FACE_OUTER_BOUND('',#14854,.T.);
#8698=FACE_OUTER_BOUND('',#14855,.T.);
#8699=FACE_OUTER_BOUND('',#14856,.T.);
#8700=FACE_OUTER_BOUND('',#14857,.T.);
#8701=FACE_OUTER_BOUND('',#14858,.T.);
#8702=FACE_OUTER_BOUND('',#14859,.T.);
#8703=FACE_OUTER_BOUND('',#14860,.T.);
#8704=FACE_OUTER_BOUND('',#14861,.T.);
#8705=FACE_OUTER_BOUND('',#14862,.T.);
#8706=FACE_OUTER_BOUND('',#14863,.T.);
#8707=FACE_OUTER_BOUND('',#14864,.T.);
#8708=FACE_OUTER_BOUND('',#14865,.T.);
#8709=FACE_OUTER_BOUND('',#14866,.T.);
#8710=FACE_OUTER_BOUND('',#14867,.T.);
#8711=FACE_OUTER_BOUND('',#14868,.T.);
#8712=FACE_OUTER_BOUND('',#14869,.T.);
#8713=FACE_OUTER_BOUND('',#14870,.T.);
#8714=FACE_OUTER_BOUND('',#14871,.T.);
#8715=FACE_OUTER_BOUND('',#14872,.T.);
#8716=FACE_OUTER_BOUND('',#14873,.T.);
#8717=FACE_OUTER_BOUND('',#14874,.T.);
#8718=FACE_OUTER_BOUND('',#14875,.T.);
#8719=FACE_OUTER_BOUND('',#14876,.T.);
#8720=FACE_OUTER_BOUND('',#14877,.T.);
#8721=FACE_OUTER_BOUND('',#14878,.T.);
#8722=FACE_OUTER_BOUND('',#14879,.T.);
#8723=FACE_OUTER_BOUND('',#14880,.T.);
#8724=FACE_OUTER_BOUND('',#14881,.T.);
#8725=FACE_OUTER_BOUND('',#14882,.T.);
#8726=FACE_OUTER_BOUND('',#14883,.T.);
#8727=FACE_OUTER_BOUND('',#14884,.T.);
#8728=FACE_OUTER_BOUND('',#14885,.T.);
#8729=FACE_OUTER_BOUND('',#14886,.T.);
#8730=FACE_OUTER_BOUND('',#14887,.T.);
#8731=FACE_OUTER_BOUND('',#14888,.T.);
#8732=FACE_OUTER_BOUND('',#14889,.T.);
#8733=FACE_OUTER_BOUND('',#14890,.T.);
#8734=FACE_OUTER_BOUND('',#14891,.T.);
#8735=FACE_OUTER_BOUND('',#14892,.T.);
#8736=FACE_OUTER_BOUND('',#14893,.T.);
#8737=FACE_OUTER_BOUND('',#14894,.T.);
#8738=FACE_OUTER_BOUND('',#14895,.T.);
#8739=FACE_OUTER_BOUND('',#14896,.T.);
#8740=FACE_OUTER_BOUND('',#14897,.T.);
#8741=FACE_OUTER_BOUND('',#14898,.T.);
#8742=FACE_OUTER_BOUND('',#14899,.T.);
#8743=FACE_OUTER_BOUND('',#14900,.T.);
#8744=FACE_OUTER_BOUND('',#14901,.T.);
#8745=FACE_OUTER_BOUND('',#14902,.T.);
#8746=FACE_OUTER_BOUND('',#14903,.T.);
#8747=FACE_OUTER_BOUND('',#14904,.T.);
#8748=FACE_OUTER_BOUND('',#14905,.T.);
#8749=FACE_OUTER_BOUND('',#14906,.T.);
#8750=FACE_OUTER_BOUND('',#14907,.T.);
#8751=FACE_OUTER_BOUND('',#14908,.T.);
#8752=FACE_OUTER_BOUND('',#14909,.T.);
#8753=FACE_OUTER_BOUND('',#14910,.T.);
#8754=FACE_OUTER_BOUND('',#14911,.T.);
#8755=FACE_OUTER_BOUND('',#14912,.T.);
#8756=FACE_OUTER_BOUND('',#14913,.T.);
#8757=FACE_OUTER_BOUND('',#14914,.T.);
#8758=FACE_OUTER_BOUND('',#14915,.T.);
#8759=FACE_OUTER_BOUND('',#14916,.T.);
#8760=FACE_OUTER_BOUND('',#14917,.T.);
#8761=FACE_OUTER_BOUND('',#14918,.T.);
#8762=FACE_OUTER_BOUND('',#14919,.T.);
#8763=FACE_OUTER_BOUND('',#14920,.T.);
#8764=FACE_OUTER_BOUND('',#14921,.T.);
#8765=FACE_OUTER_BOUND('',#14922,.T.);
#8766=FACE_OUTER_BOUND('',#14923,.T.);
#8767=FACE_OUTER_BOUND('',#14924,.T.);
#8768=FACE_OUTER_BOUND('',#14925,.T.);
#8769=FACE_OUTER_BOUND('',#14926,.T.);
#8770=FACE_OUTER_BOUND('',#14927,.T.);
#8771=FACE_OUTER_BOUND('',#14928,.T.);
#8772=FACE_OUTER_BOUND('',#14929,.T.);
#8773=FACE_OUTER_BOUND('',#14930,.T.);
#8774=FACE_OUTER_BOUND('',#14931,.T.);
#8775=FACE_OUTER_BOUND('',#14932,.T.);
#8776=FACE_OUTER_BOUND('',#14933,.T.);
#8777=FACE_OUTER_BOUND('',#14934,.T.);
#8778=FACE_OUTER_BOUND('',#14935,.T.);
#8779=FACE_OUTER_BOUND('',#14936,.T.);
#8780=FACE_OUTER_BOUND('',#14937,.T.);
#8781=FACE_OUTER_BOUND('',#14938,.T.);
#8782=FACE_OUTER_BOUND('',#14939,.T.);
#8783=FACE_OUTER_BOUND('',#14940,.T.);
#8784=FACE_OUTER_BOUND('',#14941,.T.);
#8785=FACE_OUTER_BOUND('',#14942,.T.);
#8786=FACE_OUTER_BOUND('',#14943,.T.);
#8787=FACE_OUTER_BOUND('',#14944,.T.);
#8788=FACE_OUTER_BOUND('',#14945,.T.);
#8789=FACE_OUTER_BOUND('',#14946,.T.);
#8790=FACE_OUTER_BOUND('',#14947,.T.);
#8791=FACE_OUTER_BOUND('',#14948,.T.);
#8792=FACE_OUTER_BOUND('',#14949,.T.);
#8793=FACE_OUTER_BOUND('',#14950,.T.);
#8794=FACE_OUTER_BOUND('',#14951,.T.);
#8795=FACE_OUTER_BOUND('',#14952,.T.);
#8796=FACE_OUTER_BOUND('',#14953,.T.);
#8797=FACE_OUTER_BOUND('',#14954,.T.);
#8798=FACE_OUTER_BOUND('',#14955,.T.);
#8799=FACE_OUTER_BOUND('',#14956,.T.);
#8800=FACE_OUTER_BOUND('',#14957,.T.);
#8801=FACE_OUTER_BOUND('',#14958,.T.);
#8802=FACE_OUTER_BOUND('',#14959,.T.);
#8803=FACE_OUTER_BOUND('',#14960,.T.);
#8804=FACE_OUTER_BOUND('',#14961,.T.);
#8805=FACE_OUTER_BOUND('',#14962,.T.);
#8806=FACE_OUTER_BOUND('',#14963,.T.);
#8807=FACE_OUTER_BOUND('',#14964,.T.);
#8808=FACE_OUTER_BOUND('',#14965,.T.);
#8809=FACE_OUTER_BOUND('',#14966,.T.);
#8810=FACE_OUTER_BOUND('',#14967,.T.);
#8811=FACE_OUTER_BOUND('',#14968,.T.);
#8812=FACE_OUTER_BOUND('',#14969,.T.);
#8813=FACE_OUTER_BOUND('',#14970,.T.);
#8814=FACE_OUTER_BOUND('',#14971,.T.);
#8815=FACE_OUTER_BOUND('',#14972,.T.);
#8816=FACE_OUTER_BOUND('',#14973,.T.);
#8817=FACE_OUTER_BOUND('',#14974,.T.);
#8818=FACE_OUTER_BOUND('',#14975,.T.);
#8819=FACE_OUTER_BOUND('',#14976,.T.);
#8820=FACE_OUTER_BOUND('',#14977,.T.);
#8821=FACE_OUTER_BOUND('',#14978,.T.);
#8822=FACE_OUTER_BOUND('',#14979,.T.);
#8823=FACE_OUTER_BOUND('',#14980,.T.);
#8824=FACE_OUTER_BOUND('',#14981,.T.);
#8825=FACE_OUTER_BOUND('',#14982,.T.);
#8826=FACE_OUTER_BOUND('',#14983,.T.);
#8827=FACE_OUTER_BOUND('',#14984,.T.);
#8828=FACE_OUTER_BOUND('',#14985,.T.);
#8829=FACE_OUTER_BOUND('',#14986,.T.);
#8830=FACE_OUTER_BOUND('',#14987,.T.);
#8831=FACE_OUTER_BOUND('',#14988,.T.);
#8832=FACE_OUTER_BOUND('',#14989,.T.);
#8833=FACE_OUTER_BOUND('',#14990,.T.);
#8834=FACE_OUTER_BOUND('',#14991,.T.);
#8835=FACE_OUTER_BOUND('',#14992,.T.);
#8836=FACE_OUTER_BOUND('',#14993,.T.);
#8837=FACE_OUTER_BOUND('',#14994,.T.);
#8838=FACE_OUTER_BOUND('',#14995,.T.);
#8839=FACE_OUTER_BOUND('',#14996,.T.);
#8840=FACE_OUTER_BOUND('',#14997,.T.);
#8841=FACE_OUTER_BOUND('',#14998,.T.);
#8842=FACE_OUTER_BOUND('',#14999,.T.);
#8843=FACE_OUTER_BOUND('',#15000,.T.);
#8844=FACE_OUTER_BOUND('',#15001,.T.);
#8845=FACE_OUTER_BOUND('',#15002,.T.);
#8846=FACE_OUTER_BOUND('',#15003,.T.);
#8847=FACE_OUTER_BOUND('',#15004,.T.);
#8848=FACE_OUTER_BOUND('',#15005,.T.);
#8849=FACE_OUTER_BOUND('',#15006,.T.);
#8850=FACE_OUTER_BOUND('',#15007,.T.);
#8851=FACE_OUTER_BOUND('',#15008,.T.);
#8852=FACE_OUTER_BOUND('',#15009,.T.);
#8853=FACE_OUTER_BOUND('',#15010,.T.);
#8854=FACE_OUTER_BOUND('',#15011,.T.);
#8855=FACE_OUTER_BOUND('',#15012,.T.);
#8856=FACE_OUTER_BOUND('',#15013,.T.);
#8857=FACE_OUTER_BOUND('',#15014,.T.);
#8858=FACE_OUTER_BOUND('',#15015,.T.);
#8859=FACE_OUTER_BOUND('',#15016,.T.);
#8860=FACE_OUTER_BOUND('',#15017,.T.);
#8861=FACE_OUTER_BOUND('',#15018,.T.);
#8862=FACE_OUTER_BOUND('',#15019,.T.);
#8863=FACE_OUTER_BOUND('',#15020,.T.);
#8864=FACE_OUTER_BOUND('',#15021,.T.);
#8865=FACE_OUTER_BOUND('',#15022,.T.);
#8866=FACE_OUTER_BOUND('',#15023,.T.);
#8867=FACE_OUTER_BOUND('',#15024,.T.);
#8868=FACE_OUTER_BOUND('',#15025,.T.);
#8869=FACE_OUTER_BOUND('',#15026,.T.);
#8870=FACE_OUTER_BOUND('',#15027,.T.);
#8871=FACE_OUTER_BOUND('',#15028,.T.);
#8872=FACE_OUTER_BOUND('',#15029,.T.);
#8873=FACE_OUTER_BOUND('',#15030,.T.);
#8874=FACE_OUTER_BOUND('',#15031,.T.);
#8875=FACE_OUTER_BOUND('',#15032,.T.);
#8876=FACE_OUTER_BOUND('',#15033,.T.);
#8877=FACE_OUTER_BOUND('',#15034,.T.);
#8878=FACE_OUTER_BOUND('',#15035,.T.);
#8879=FACE_OUTER_BOUND('',#15036,.T.);
#8880=FACE_OUTER_BOUND('',#15037,.T.);
#8881=FACE_OUTER_BOUND('',#15038,.T.);
#8882=FACE_OUTER_BOUND('',#15039,.T.);
#8883=FACE_OUTER_BOUND('',#15040,.T.);
#8884=FACE_OUTER_BOUND('',#15041,.T.);
#8885=FACE_OUTER_BOUND('',#15042,.T.);
#8886=FACE_OUTER_BOUND('',#15043,.T.);
#8887=FACE_OUTER_BOUND('',#15044,.T.);
#8888=FACE_OUTER_BOUND('',#15045,.T.);
#8889=FACE_OUTER_BOUND('',#15046,.T.);
#8890=FACE_OUTER_BOUND('',#15047,.T.);
#8891=FACE_OUTER_BOUND('',#15048,.T.);
#8892=FACE_OUTER_BOUND('',#15049,.T.);
#8893=FACE_OUTER_BOUND('',#15050,.T.);
#8894=FACE_OUTER_BOUND('',#15051,.T.);
#8895=FACE_OUTER_BOUND('',#15052,.T.);
#8896=FACE_OUTER_BOUND('',#15053,.T.);
#8897=FACE_OUTER_BOUND('',#15054,.T.);
#8898=FACE_OUTER_BOUND('',#15055,.T.);
#8899=FACE_OUTER_BOUND('',#15056,.T.);
#8900=FACE_OUTER_BOUND('',#15057,.T.);
#8901=FACE_OUTER_BOUND('',#15058,.T.);
#8902=FACE_OUTER_BOUND('',#15059,.T.);
#8903=FACE_OUTER_BOUND('',#15060,.T.);
#8904=FACE_OUTER_BOUND('',#15061,.T.);
#8905=FACE_OUTER_BOUND('',#15062,.T.);
#8906=FACE_OUTER_BOUND('',#15063,.T.);
#8907=FACE_OUTER_BOUND('',#15064,.T.);
#8908=FACE_OUTER_BOUND('',#15065,.T.);
#8909=FACE_OUTER_BOUND('',#15066,.T.);
#8910=FACE_OUTER_BOUND('',#15067,.T.);
#8911=FACE_OUTER_BOUND('',#15068,.T.);
#8912=FACE_OUTER_BOUND('',#15069,.T.);
#8913=FACE_OUTER_BOUND('',#15070,.T.);
#8914=FACE_OUTER_BOUND('',#15071,.T.);
#8915=FACE_OUTER_BOUND('',#15072,.T.);
#8916=FACE_OUTER_BOUND('',#15073,.T.);
#8917=FACE_OUTER_BOUND('',#15074,.T.);
#8918=FACE_OUTER_BOUND('',#15075,.T.);
#8919=FACE_OUTER_BOUND('',#15076,.T.);
#8920=FACE_OUTER_BOUND('',#15077,.T.);
#8921=FACE_OUTER_BOUND('',#15078,.T.);
#8922=FACE_OUTER_BOUND('',#15079,.T.);
#8923=FACE_OUTER_BOUND('',#15080,.T.);
#8924=FACE_OUTER_BOUND('',#15081,.T.);
#8925=FACE_OUTER_BOUND('',#15082,.T.);
#8926=FACE_OUTER_BOUND('',#15083,.T.);
#8927=FACE_OUTER_BOUND('',#15084,.T.);
#8928=FACE_OUTER_BOUND('',#15085,.T.);
#8929=FACE_OUTER_BOUND('',#15086,.T.);
#8930=FACE_OUTER_BOUND('',#15087,.T.);
#8931=FACE_OUTER_BOUND('',#15088,.T.);
#8932=FACE_OUTER_BOUND('',#15089,.T.);
#8933=FACE_OUTER_BOUND('',#15090,.T.);
#8934=FACE_OUTER_BOUND('',#15091,.T.);
#8935=FACE_OUTER_BOUND('',#15092,.T.);
#8936=FACE_OUTER_BOUND('',#15093,.T.);
#8937=FACE_OUTER_BOUND('',#15094,.T.);
#8938=FACE_OUTER_BOUND('',#15095,.T.);
#8939=FACE_OUTER_BOUND('',#15096,.T.);
#8940=FACE_OUTER_BOUND('',#15097,.T.);
#8941=FACE_OUTER_BOUND('',#15098,.T.);
#8942=FACE_OUTER_BOUND('',#15099,.T.);
#8943=FACE_OUTER_BOUND('',#15100,.T.);
#8944=FACE_OUTER_BOUND('',#15101,.T.);
#8945=FACE_OUTER_BOUND('',#15102,.T.);
#8946=FACE_OUTER_BOUND('',#15103,.T.);
#8947=FACE_OUTER_BOUND('',#15104,.T.);
#8948=FACE_OUTER_BOUND('',#15105,.T.);
#8949=FACE_OUTER_BOUND('',#15106,.T.);
#8950=FACE_OUTER_BOUND('',#15107,.T.);
#8951=FACE_OUTER_BOUND('',#15108,.T.);
#8952=FACE_OUTER_BOUND('',#15109,.T.);
#8953=FACE_OUTER_BOUND('',#15110,.T.);
#8954=FACE_OUTER_BOUND('',#15111,.T.);
#8955=FACE_OUTER_BOUND('',#15112,.T.);
#8956=FACE_OUTER_BOUND('',#15113,.T.);
#8957=FACE_OUTER_BOUND('',#15114,.T.);
#8958=FACE_OUTER_BOUND('',#15115,.T.);
#8959=FACE_OUTER_BOUND('',#15116,.T.);
#8960=FACE_OUTER_BOUND('',#15117,.T.);
#8961=FACE_OUTER_BOUND('',#15118,.T.);
#8962=FACE_OUTER_BOUND('',#15119,.T.);
#8963=FACE_OUTER_BOUND('',#15120,.T.);
#8964=FACE_OUTER_BOUND('',#15121,.T.);
#8965=FACE_OUTER_BOUND('',#15122,.T.);
#8966=FACE_OUTER_BOUND('',#15123,.T.);
#8967=FACE_OUTER_BOUND('',#15124,.T.);
#8968=FACE_OUTER_BOUND('',#15125,.T.);
#8969=FACE_OUTER_BOUND('',#15126,.T.);
#8970=FACE_OUTER_BOUND('',#15127,.T.);
#8971=FACE_OUTER_BOUND('',#15128,.T.);
#8972=FACE_OUTER_BOUND('',#15129,.T.);
#8973=FACE_OUTER_BOUND('',#15130,.T.);
#8974=FACE_OUTER_BOUND('',#15131,.T.);
#8975=FACE_OUTER_BOUND('',#15132,.T.);
#8976=FACE_OUTER_BOUND('',#15133,.T.);
#8977=FACE_OUTER_BOUND('',#15134,.T.);
#8978=FACE_OUTER_BOUND('',#15135,.T.);
#8979=FACE_OUTER_BOUND('',#15136,.T.);
#8980=FACE_OUTER_BOUND('',#15137,.T.);
#8981=FACE_OUTER_BOUND('',#15138,.T.);
#8982=FACE_OUTER_BOUND('',#15139,.T.);
#8983=FACE_OUTER_BOUND('',#15140,.T.);
#8984=FACE_OUTER_BOUND('',#15141,.T.);
#8985=FACE_OUTER_BOUND('',#15142,.T.);
#8986=FACE_OUTER_BOUND('',#15143,.T.);
#8987=FACE_OUTER_BOUND('',#15144,.T.);
#8988=FACE_OUTER_BOUND('',#15145,.T.);
#8989=FACE_OUTER_BOUND('',#15146,.T.);
#8990=FACE_OUTER_BOUND('',#15147,.T.);
#8991=FACE_OUTER_BOUND('',#15148,.T.);
#8992=FACE_OUTER_BOUND('',#15149,.T.);
#8993=FACE_OUTER_BOUND('',#15150,.T.);
#8994=FACE_OUTER_BOUND('',#15151,.T.);
#8995=FACE_OUTER_BOUND('',#15152,.T.);
#8996=FACE_OUTER_BOUND('',#15153,.T.);
#8997=FACE_OUTER_BOUND('',#15154,.T.);
#8998=FACE_OUTER_BOUND('',#15155,.T.);
#8999=FACE_OUTER_BOUND('',#15156,.T.);
#9000=FACE_OUTER_BOUND('',#15157,.T.);
#9001=FACE_OUTER_BOUND('',#15158,.T.);
#9002=FACE_OUTER_BOUND('',#15159,.T.);
#9003=FACE_OUTER_BOUND('',#15160,.T.);
#9004=FACE_OUTER_BOUND('',#15161,.T.);
#9005=FACE_OUTER_BOUND('',#15162,.T.);
#9006=FACE_OUTER_BOUND('',#15163,.T.);
#9007=FACE_OUTER_BOUND('',#15164,.T.);
#9008=FACE_OUTER_BOUND('',#15165,.T.);
#9009=FACE_OUTER_BOUND('',#15166,.T.);
#9010=FACE_OUTER_BOUND('',#15167,.T.);
#9011=FACE_OUTER_BOUND('',#15168,.T.);
#9012=FACE_OUTER_BOUND('',#15169,.T.);
#9013=FACE_OUTER_BOUND('',#15170,.T.);
#9014=FACE_OUTER_BOUND('',#15171,.T.);
#9015=FACE_OUTER_BOUND('',#15172,.T.);
#9016=FACE_OUTER_BOUND('',#15173,.T.);
#9017=FACE_OUTER_BOUND('',#15174,.T.);
#9018=FACE_OUTER_BOUND('',#15175,.T.);
#9019=FACE_OUTER_BOUND('',#15176,.T.);
#9020=FACE_OUTER_BOUND('',#15177,.T.);
#9021=FACE_OUTER_BOUND('',#15178,.T.);
#9022=FACE_OUTER_BOUND('',#15179,.T.);
#9023=FACE_OUTER_BOUND('',#15180,.T.);
#9024=FACE_OUTER_BOUND('',#15181,.T.);
#9025=FACE_OUTER_BOUND('',#15182,.T.);
#9026=FACE_OUTER_BOUND('',#15183,.T.);
#9027=FACE_OUTER_BOUND('',#15184,.T.);
#9028=FACE_OUTER_BOUND('',#15185,.T.);
#9029=FACE_OUTER_BOUND('',#15186,.T.);
#9030=FACE_OUTER_BOUND('',#15187,.T.);
#9031=FACE_OUTER_BOUND('',#15188,.T.);
#9032=FACE_OUTER_BOUND('',#15189,.T.);
#9033=FACE_OUTER_BOUND('',#15190,.T.);
#9034=FACE_OUTER_BOUND('',#15191,.T.);
#9035=FACE_OUTER_BOUND('',#15192,.T.);
#9036=FACE_OUTER_BOUND('',#15193,.T.);
#9037=FACE_OUTER_BOUND('',#15194,.T.);
#9038=FACE_OUTER_BOUND('',#15195,.T.);
#9039=FACE_OUTER_BOUND('',#15196,.T.);
#9040=FACE_OUTER_BOUND('',#15197,.T.);
#9041=FACE_OUTER_BOUND('',#15198,.T.);
#9042=FACE_OUTER_BOUND('',#15199,.T.);
#9043=FACE_OUTER_BOUND('',#15200,.T.);
#9044=FACE_OUTER_BOUND('',#15201,.T.);
#9045=FACE_OUTER_BOUND('',#15202,.T.);
#9046=FACE_OUTER_BOUND('',#15203,.T.);
#9047=FACE_OUTER_BOUND('',#15204,.T.);
#9048=FACE_OUTER_BOUND('',#15205,.T.);
#9049=FACE_OUTER_BOUND('',#15206,.T.);
#9050=FACE_OUTER_BOUND('',#15207,.T.);
#9051=FACE_OUTER_BOUND('',#15208,.T.);
#9052=FACE_OUTER_BOUND('',#15209,.T.);
#9053=FACE_OUTER_BOUND('',#15210,.T.);
#9054=FACE_OUTER_BOUND('',#15211,.T.);
#9055=FACE_OUTER_BOUND('',#15212,.T.);
#9056=FACE_OUTER_BOUND('',#15213,.T.);
#9057=FACE_OUTER_BOUND('',#15214,.T.);
#9058=FACE_OUTER_BOUND('',#15215,.T.);
#9059=FACE_OUTER_BOUND('',#15216,.T.);
#9060=FACE_OUTER_BOUND('',#15217,.T.);
#9061=FACE_OUTER_BOUND('',#15218,.T.);
#9062=FACE_OUTER_BOUND('',#15219,.T.);
#9063=FACE_OUTER_BOUND('',#15220,.T.);
#9064=FACE_OUTER_BOUND('',#15221,.T.);
#9065=FACE_OUTER_BOUND('',#15222,.T.);
#9066=FACE_OUTER_BOUND('',#15223,.T.);
#9067=FACE_OUTER_BOUND('',#15224,.T.);
#9068=FACE_OUTER_BOUND('',#15225,.T.);
#9069=FACE_OUTER_BOUND('',#15226,.T.);
#9070=FACE_OUTER_BOUND('',#15227,.T.);
#9071=FACE_OUTER_BOUND('',#15228,.T.);
#9072=FACE_OUTER_BOUND('',#15229,.T.);
#9073=FACE_OUTER_BOUND('',#15230,.T.);
#9074=FACE_OUTER_BOUND('',#15231,.T.);
#9075=FACE_OUTER_BOUND('',#15232,.T.);
#9076=FACE_OUTER_BOUND('',#15233,.T.);
#9077=FACE_OUTER_BOUND('',#15234,.T.);
#9078=FACE_OUTER_BOUND('',#15235,.T.);
#9079=FACE_OUTER_BOUND('',#15236,.T.);
#9080=FACE_OUTER_BOUND('',#15237,.T.);
#9081=FACE_OUTER_BOUND('',#15238,.T.);
#9082=FACE_OUTER_BOUND('',#15239,.T.);
#9083=FACE_OUTER_BOUND('',#15240,.T.);
#9084=FACE_OUTER_BOUND('',#15241,.T.);
#9085=FACE_OUTER_BOUND('',#15242,.T.);
#9086=FACE_OUTER_BOUND('',#15243,.T.);
#9087=FACE_OUTER_BOUND('',#15244,.T.);
#9088=FACE_OUTER_BOUND('',#15245,.T.);
#9089=FACE_OUTER_BOUND('',#15246,.T.);
#9090=FACE_OUTER_BOUND('',#15247,.T.);
#9091=FACE_OUTER_BOUND('',#15248,.T.);
#9092=FACE_OUTER_BOUND('',#15249,.T.);
#9093=FACE_OUTER_BOUND('',#15250,.T.);
#9094=FACE_OUTER_BOUND('',#15251,.T.);
#9095=FACE_OUTER_BOUND('',#15252,.T.);
#9096=FACE_OUTER_BOUND('',#15253,.T.);
#9097=FACE_OUTER_BOUND('',#15254,.T.);
#9098=FACE_OUTER_BOUND('',#15255,.T.);
#9099=FACE_OUTER_BOUND('',#15256,.T.);
#9100=FACE_OUTER_BOUND('',#15257,.T.);
#9101=FACE_OUTER_BOUND('',#15258,.T.);
#9102=FACE_OUTER_BOUND('',#15259,.T.);
#9103=FACE_OUTER_BOUND('',#15260,.T.);
#9104=FACE_OUTER_BOUND('',#15261,.T.);
#9105=FACE_OUTER_BOUND('',#15262,.T.);
#9106=FACE_OUTER_BOUND('',#15263,.T.);
#9107=FACE_OUTER_BOUND('',#15264,.T.);
#9108=FACE_OUTER_BOUND('',#15265,.T.);
#9109=FACE_OUTER_BOUND('',#15266,.T.);
#9110=FACE_OUTER_BOUND('',#15267,.T.);
#9111=FACE_OUTER_BOUND('',#15268,.T.);
#9112=FACE_OUTER_BOUND('',#15269,.T.);
#9113=FACE_OUTER_BOUND('',#15270,.T.);
#9114=FACE_OUTER_BOUND('',#15271,.T.);
#9115=FACE_OUTER_BOUND('',#15272,.T.);
#9116=FACE_OUTER_BOUND('',#15273,.T.);
#9117=FACE_OUTER_BOUND('',#15274,.T.);
#9118=FACE_OUTER_BOUND('',#15275,.T.);
#9119=FACE_OUTER_BOUND('',#15276,.T.);
#9120=FACE_OUTER_BOUND('',#15277,.T.);
#9121=FACE_OUTER_BOUND('',#15278,.T.);
#9122=FACE_OUTER_BOUND('',#15279,.T.);
#9123=FACE_OUTER_BOUND('',#15280,.T.);
#9124=FACE_OUTER_BOUND('',#15281,.T.);
#9125=FACE_OUTER_BOUND('',#15282,.T.);
#9126=FACE_OUTER_BOUND('',#15283,.T.);
#9127=FACE_OUTER_BOUND('',#15284,.T.);
#9128=FACE_OUTER_BOUND('',#15285,.T.);
#9129=FACE_OUTER_BOUND('',#15286,.T.);
#9130=FACE_OUTER_BOUND('',#15287,.T.);
#9131=FACE_OUTER_BOUND('',#15288,.T.);
#9132=FACE_OUTER_BOUND('',#15289,.T.);
#9133=FACE_OUTER_BOUND('',#15290,.T.);
#9134=FACE_OUTER_BOUND('',#15291,.T.);
#9135=FACE_OUTER_BOUND('',#15292,.T.);
#9136=FACE_OUTER_BOUND('',#15293,.T.);
#9137=FACE_OUTER_BOUND('',#15294,.T.);
#9138=FACE_OUTER_BOUND('',#15295,.T.);
#9139=FACE_OUTER_BOUND('',#15296,.T.);
#9140=FACE_OUTER_BOUND('',#15297,.T.);
#9141=FACE_OUTER_BOUND('',#15298,.T.);
#9142=FACE_OUTER_BOUND('',#15299,.T.);
#9143=FACE_OUTER_BOUND('',#15300,.T.);
#9144=FACE_OUTER_BOUND('',#15301,.T.);
#9145=FACE_OUTER_BOUND('',#15302,.T.);
#9146=FACE_OUTER_BOUND('',#15303,.T.);
#9147=FACE_OUTER_BOUND('',#15304,.T.);
#9148=FACE_OUTER_BOUND('',#15305,.T.);
#9149=FACE_OUTER_BOUND('',#15306,.T.);
#9150=FACE_OUTER_BOUND('',#15307,.T.);
#9151=FACE_OUTER_BOUND('',#15308,.T.);
#9152=FACE_OUTER_BOUND('',#15309,.T.);
#9153=FACE_OUTER_BOUND('',#15310,.T.);
#9154=FACE_OUTER_BOUND('',#15311,.T.);
#9155=FACE_OUTER_BOUND('',#15312,.T.);
#9156=FACE_OUTER_BOUND('',#15313,.T.);
#9157=FACE_OUTER_BOUND('',#15314,.T.);
#9158=FACE_OUTER_BOUND('',#15315,.T.);
#9159=FACE_OUTER_BOUND('',#15316,.T.);
#9160=FACE_OUTER_BOUND('',#15317,.T.);
#9161=FACE_OUTER_BOUND('',#15318,.T.);
#9162=FACE_OUTER_BOUND('',#15319,.T.);
#9163=FACE_OUTER_BOUND('',#15320,.T.);
#9164=FACE_OUTER_BOUND('',#15321,.T.);
#9165=FACE_OUTER_BOUND('',#15322,.T.);
#9166=FACE_OUTER_BOUND('',#15323,.T.);
#9167=FACE_OUTER_BOUND('',#15324,.T.);
#9168=FACE_OUTER_BOUND('',#15325,.T.);
#9169=FACE_OUTER_BOUND('',#15326,.T.);
#9170=FACE_OUTER_BOUND('',#15327,.T.);
#9171=FACE_OUTER_BOUND('',#15328,.T.);
#9172=FACE_OUTER_BOUND('',#15329,.T.);
#9173=FACE_OUTER_BOUND('',#15330,.T.);
#9174=FACE_OUTER_BOUND('',#15331,.T.);
#9175=FACE_OUTER_BOUND('',#15332,.T.);
#9176=FACE_OUTER_BOUND('',#15333,.T.);
#9177=FACE_OUTER_BOUND('',#15334,.T.);
#9178=FACE_OUTER_BOUND('',#15335,.T.);
#9179=FACE_OUTER_BOUND('',#15336,.T.);
#9180=FACE_OUTER_BOUND('',#15337,.T.);
#9181=FACE_OUTER_BOUND('',#15338,.T.);
#9182=FACE_OUTER_BOUND('',#15339,.T.);
#9183=FACE_OUTER_BOUND('',#15340,.T.);
#9184=FACE_OUTER_BOUND('',#15341,.T.);
#9185=FACE_OUTER_BOUND('',#15342,.T.);
#9186=FACE_OUTER_BOUND('',#15343,.T.);
#9187=FACE_OUTER_BOUND('',#15344,.T.);
#9188=FACE_OUTER_BOUND('',#15345,.T.);
#9189=FACE_OUTER_BOUND('',#15346,.T.);
#9190=FACE_OUTER_BOUND('',#15347,.T.);
#9191=FACE_OUTER_BOUND('',#15348,.T.);
#9192=FACE_OUTER_BOUND('',#15349,.T.);
#9193=FACE_OUTER_BOUND('',#15350,.T.);
#9194=FACE_OUTER_BOUND('',#15351,.T.);
#9195=FACE_OUTER_BOUND('',#15352,.T.);
#9196=FACE_OUTER_BOUND('',#15353,.T.);
#9197=FACE_OUTER_BOUND('',#15354,.T.);
#9198=FACE_OUTER_BOUND('',#15355,.T.);
#9199=FACE_OUTER_BOUND('',#15356,.T.);
#9200=FACE_OUTER_BOUND('',#15357,.T.);
#9201=FACE_OUTER_BOUND('',#15358,.T.);
#9202=FACE_OUTER_BOUND('',#15359,.T.);
#9203=FACE_OUTER_BOUND('',#15360,.T.);
#9204=FACE_OUTER_BOUND('',#15361,.T.);
#9205=FACE_OUTER_BOUND('',#15362,.T.);
#9206=FACE_OUTER_BOUND('',#15363,.T.);
#9207=FACE_OUTER_BOUND('',#15364,.T.);
#9208=FACE_OUTER_BOUND('',#15365,.T.);
#9209=FACE_OUTER_BOUND('',#15366,.T.);
#9210=FACE_OUTER_BOUND('',#15367,.T.);
#9211=FACE_OUTER_BOUND('',#15368,.T.);
#9212=FACE_OUTER_BOUND('',#15369,.T.);
#9213=FACE_OUTER_BOUND('',#15370,.T.);
#9214=FACE_OUTER_BOUND('',#15371,.T.);
#9215=FACE_OUTER_BOUND('',#15372,.T.);
#9216=FACE_OUTER_BOUND('',#15373,.T.);
#9217=FACE_OUTER_BOUND('',#15374,.T.);
#9218=FACE_OUTER_BOUND('',#15375,.T.);
#9219=FACE_OUTER_BOUND('',#15376,.T.);
#9220=FACE_OUTER_BOUND('',#15377,.T.);
#9221=FACE_OUTER_BOUND('',#15378,.T.);
#9222=FACE_OUTER_BOUND('',#15379,.T.);
#9223=FACE_OUTER_BOUND('',#15380,.T.);
#9224=FACE_OUTER_BOUND('',#15381,.T.);
#9225=FACE_OUTER_BOUND('',#15382,.T.);
#9226=FACE_OUTER_BOUND('',#15383,.T.);
#9227=FACE_OUTER_BOUND('',#15384,.T.);
#9228=FACE_OUTER_BOUND('',#15385,.T.);
#9229=FACE_OUTER_BOUND('',#15386,.T.);
#9230=FACE_OUTER_BOUND('',#15387,.T.);
#9231=FACE_OUTER_BOUND('',#15388,.T.);
#9232=FACE_OUTER_BOUND('',#15389,.T.);
#9233=FACE_OUTER_BOUND('',#15390,.T.);
#9234=FACE_OUTER_BOUND('',#15391,.T.);
#9235=FACE_OUTER_BOUND('',#15392,.T.);
#9236=FACE_OUTER_BOUND('',#15393,.T.);
#9237=FACE_OUTER_BOUND('',#15394,.T.);
#9238=FACE_OUTER_BOUND('',#15395,.T.);
#9239=FACE_OUTER_BOUND('',#15396,.T.);
#9240=FACE_OUTER_BOUND('',#15397,.T.);
#9241=FACE_OUTER_BOUND('',#15398,.T.);
#9242=FACE_OUTER_BOUND('',#15399,.T.);
#9243=FACE_OUTER_BOUND('',#15400,.T.);
#9244=FACE_OUTER_BOUND('',#15401,.T.);
#9245=FACE_OUTER_BOUND('',#15402,.T.);
#9246=FACE_OUTER_BOUND('',#15403,.T.);
#9247=FACE_OUTER_BOUND('',#15404,.T.);
#9248=FACE_OUTER_BOUND('',#15405,.T.);
#9249=FACE_OUTER_BOUND('',#15406,.T.);
#9250=FACE_OUTER_BOUND('',#15407,.T.);
#9251=FACE_OUTER_BOUND('',#15408,.T.);
#9252=FACE_OUTER_BOUND('',#15409,.T.);
#9253=FACE_OUTER_BOUND('',#15410,.T.);
#9254=FACE_OUTER_BOUND('',#15411,.T.);
#9255=FACE_OUTER_BOUND('',#15412,.T.);
#9256=FACE_OUTER_BOUND('',#15413,.T.);
#9257=FACE_OUTER_BOUND('',#15414,.T.);
#9258=FACE_OUTER_BOUND('',#15415,.T.);
#9259=FACE_OUTER_BOUND('',#15416,.T.);
#9260=FACE_OUTER_BOUND('',#15417,.T.);
#9261=FACE_OUTER_BOUND('',#15418,.T.);
#9262=FACE_OUTER_BOUND('',#15419,.T.);
#9263=FACE_OUTER_BOUND('',#15420,.T.);
#9264=FACE_OUTER_BOUND('',#15421,.T.);
#9265=FACE_OUTER_BOUND('',#15422,.T.);
#9266=FACE_OUTER_BOUND('',#15423,.T.);
#9267=FACE_OUTER_BOUND('',#15424,.T.);
#9268=FACE_OUTER_BOUND('',#15425,.T.);
#9269=FACE_OUTER_BOUND('',#15426,.T.);
#9270=FACE_OUTER_BOUND('',#15427,.T.);
#9271=FACE_OUTER_BOUND('',#15428,.T.);
#9272=FACE_OUTER_BOUND('',#15429,.T.);
#9273=FACE_OUTER_BOUND('',#15430,.T.);
#9274=FACE_OUTER_BOUND('',#15431,.T.);
#9275=FACE_OUTER_BOUND('',#15432,.T.);
#9276=FACE_OUTER_BOUND('',#15433,.T.);
#9277=FACE_OUTER_BOUND('',#15434,.T.);
#9278=FACE_OUTER_BOUND('',#15435,.T.);
#9279=FACE_OUTER_BOUND('',#15436,.T.);
#9280=FACE_OUTER_BOUND('',#15437,.T.);
#9281=FACE_OUTER_BOUND('',#15438,.T.);
#9282=FACE_OUTER_BOUND('',#15439,.T.);
#9283=FACE_OUTER_BOUND('',#15440,.T.);
#9284=FACE_OUTER_BOUND('',#15441,.T.);
#9285=FACE_OUTER_BOUND('',#15442,.T.);
#9286=FACE_OUTER_BOUND('',#15443,.T.);
#9287=FACE_OUTER_BOUND('',#15444,.T.);
#9288=FACE_OUTER_BOUND('',#15445,.T.);
#9289=FACE_OUTER_BOUND('',#15446,.T.);
#9290=FACE_OUTER_BOUND('',#15447,.T.);
#9291=FACE_OUTER_BOUND('',#15448,.T.);
#9292=FACE_OUTER_BOUND('',#15449,.T.);
#9293=FACE_OUTER_BOUND('',#15450,.T.);
#9294=FACE_OUTER_BOUND('',#15451,.T.);
#9295=FACE_OUTER_BOUND('',#15452,.T.);
#9296=FACE_OUTER_BOUND('',#15453,.T.);
#9297=FACE_OUTER_BOUND('',#15454,.T.);
#9298=FACE_OUTER_BOUND('',#15455,.T.);
#9299=FACE_OUTER_BOUND('',#15456,.T.);
#9300=FACE_OUTER_BOUND('',#15457,.T.);
#9301=FACE_OUTER_BOUND('',#15458,.T.);
#9302=FACE_OUTER_BOUND('',#15459,.T.);
#9303=FACE_OUTER_BOUND('',#15460,.T.);
#9304=FACE_OUTER_BOUND('',#15461,.T.);
#9305=FACE_OUTER_BOUND('',#15462,.T.);
#9306=FACE_OUTER_BOUND('',#15463,.T.);
#9307=FACE_OUTER_BOUND('',#15464,.T.);
#9308=FACE_OUTER_BOUND('',#15465,.T.);
#9309=FACE_OUTER_BOUND('',#15466,.T.);
#9310=FACE_OUTER_BOUND('',#15467,.T.);
#9311=FACE_OUTER_BOUND('',#15468,.T.);
#9312=FACE_OUTER_BOUND('',#15469,.T.);
#9313=FACE_OUTER_BOUND('',#15470,.T.);
#9314=FACE_OUTER_BOUND('',#15471,.T.);
#9315=FACE_OUTER_BOUND('',#15472,.T.);
#9316=FACE_OUTER_BOUND('',#15473,.T.);
#9317=FACE_OUTER_BOUND('',#15474,.T.);
#9318=FACE_OUTER_BOUND('',#15475,.T.);
#9319=FACE_OUTER_BOUND('',#15476,.T.);
#9320=FACE_OUTER_BOUND('',#15477,.T.);
#9321=FACE_OUTER_BOUND('',#15478,.T.);
#9322=FACE_OUTER_BOUND('',#15479,.T.);
#9323=FACE_OUTER_BOUND('',#15480,.T.);
#9324=FACE_OUTER_BOUND('',#15481,.T.);
#9325=FACE_OUTER_BOUND('',#15482,.T.);
#9326=FACE_OUTER_BOUND('',#15483,.T.);
#9327=FACE_OUTER_BOUND('',#15484,.T.);
#9328=FACE_OUTER_BOUND('',#15485,.T.);
#9329=FACE_OUTER_BOUND('',#15486,.T.);
#9330=FACE_OUTER_BOUND('',#15487,.T.);
#9331=FACE_OUTER_BOUND('',#15488,.T.);
#9332=FACE_OUTER_BOUND('',#15489,.T.);
#9333=FACE_OUTER_BOUND('',#15490,.T.);
#9334=FACE_OUTER_BOUND('',#15491,.T.);
#9335=FACE_OUTER_BOUND('',#15492,.T.);
#9336=FACE_OUTER_BOUND('',#15493,.T.);
#9337=FACE_OUTER_BOUND('',#15494,.T.);
#9338=FACE_OUTER_BOUND('',#15495,.T.);
#9339=FACE_OUTER_BOUND('',#15496,.T.);
#9340=FACE_OUTER_BOUND('',#15497,.T.);
#9341=FACE_OUTER_BOUND('',#15498,.T.);
#9342=FACE_OUTER_BOUND('',#15499,.T.);
#9343=FACE_OUTER_BOUND('',#15500,.T.);
#9344=FACE_OUTER_BOUND('',#15501,.T.);
#9345=FACE_OUTER_BOUND('',#15502,.T.);
#9346=FACE_OUTER_BOUND('',#15503,.T.);
#9347=FACE_OUTER_BOUND('',#15504,.T.);
#9348=FACE_OUTER_BOUND('',#15505,.T.);
#9349=FACE_OUTER_BOUND('',#15506,.T.);
#9350=FACE_OUTER_BOUND('',#15507,.T.);
#9351=FACE_OUTER_BOUND('',#15508,.T.);
#9352=FACE_OUTER_BOUND('',#15509,.T.);
#9353=FACE_OUTER_BOUND('',#15510,.T.);
#9354=FACE_OUTER_BOUND('',#15511,.T.);
#9355=FACE_OUTER_BOUND('',#15512,.T.);
#9356=FACE_OUTER_BOUND('',#15513,.T.);
#9357=FACE_OUTER_BOUND('',#15514,.T.);
#9358=FACE_OUTER_BOUND('',#15515,.T.);
#9359=FACE_OUTER_BOUND('',#15516,.T.);
#9360=FACE_OUTER_BOUND('',#15517,.T.);
#9361=FACE_OUTER_BOUND('',#15518,.T.);
#9362=FACE_OUTER_BOUND('',#15519,.T.);
#9363=FACE_OUTER_BOUND('',#15520,.T.);
#9364=FACE_OUTER_BOUND('',#15521,.T.);
#9365=FACE_OUTER_BOUND('',#15522,.T.);
#9366=FACE_OUTER_BOUND('',#15523,.T.);
#9367=FACE_OUTER_BOUND('',#15524,.T.);
#9368=FACE_OUTER_BOUND('',#15525,.T.);
#9369=FACE_OUTER_BOUND('',#15526,.T.);
#9370=FACE_OUTER_BOUND('',#15527,.T.);
#9371=FACE_OUTER_BOUND('',#15528,.T.);
#9372=FACE_OUTER_BOUND('',#15529,.T.);
#9373=FACE_OUTER_BOUND('',#15530,.T.);
#9374=FACE_OUTER_BOUND('',#15531,.T.);
#9375=FACE_OUTER_BOUND('',#15532,.T.);
#9376=FACE_OUTER_BOUND('',#15533,.T.);
#9377=FACE_OUTER_BOUND('',#15534,.T.);
#9378=FACE_OUTER_BOUND('',#15535,.T.);
#9379=FACE_OUTER_BOUND('',#15536,.T.);
#9380=FACE_OUTER_BOUND('',#15537,.T.);
#9381=FACE_OUTER_BOUND('',#15538,.T.);
#9382=FACE_OUTER_BOUND('',#15539,.T.);
#9383=FACE_OUTER_BOUND('',#15540,.T.);
#9384=FACE_OUTER_BOUND('',#15541,.T.);
#9385=FACE_OUTER_BOUND('',#15542,.T.);
#9386=FACE_OUTER_BOUND('',#15543,.T.);
#9387=FACE_OUTER_BOUND('',#15544,.T.);
#9388=FACE_OUTER_BOUND('',#15545,.T.);
#9389=FACE_OUTER_BOUND('',#15546,.T.);
#9390=FACE_OUTER_BOUND('',#15547,.T.);
#9391=FACE_OUTER_BOUND('',#15548,.T.);
#9392=FACE_OUTER_BOUND('',#15549,.T.);
#9393=FACE_OUTER_BOUND('',#15550,.T.);
#9394=FACE_OUTER_BOUND('',#15551,.T.);
#9395=FACE_OUTER_BOUND('',#15552,.T.);
#9396=FACE_OUTER_BOUND('',#15553,.T.);
#9397=FACE_OUTER_BOUND('',#15554,.T.);
#9398=FACE_OUTER_BOUND('',#15555,.T.);
#9399=FACE_OUTER_BOUND('',#15556,.T.);
#9400=FACE_OUTER_BOUND('',#15557,.T.);
#9401=FACE_OUTER_BOUND('',#15558,.T.);
#9402=FACE_OUTER_BOUND('',#15559,.T.);
#9403=FACE_OUTER_BOUND('',#15560,.T.);
#9404=FACE_OUTER_BOUND('',#15561,.T.);
#9405=FACE_OUTER_BOUND('',#15562,.T.);
#9406=FACE_OUTER_BOUND('',#15563,.T.);
#9407=FACE_OUTER_BOUND('',#15564,.T.);
#9408=FACE_OUTER_BOUND('',#15565,.T.);
#9409=FACE_OUTER_BOUND('',#15566,.T.);
#9410=FACE_OUTER_BOUND('',#15567,.T.);
#9411=FACE_OUTER_BOUND('',#15568,.T.);
#9412=FACE_OUTER_BOUND('',#15569,.T.);
#9413=FACE_OUTER_BOUND('',#15570,.T.);
#9414=FACE_OUTER_BOUND('',#15571,.T.);
#9415=FACE_OUTER_BOUND('',#15572,.T.);
#9416=FACE_OUTER_BOUND('',#15573,.T.);
#9417=FACE_OUTER_BOUND('',#15574,.T.);
#9418=FACE_OUTER_BOUND('',#15575,.T.);
#9419=FACE_OUTER_BOUND('',#15576,.T.);
#9420=FACE_OUTER_BOUND('',#15577,.T.);
#9421=FACE_OUTER_BOUND('',#15578,.T.);
#9422=FACE_OUTER_BOUND('',#15579,.T.);
#9423=FACE_OUTER_BOUND('',#15580,.T.);
#9424=FACE_OUTER_BOUND('',#15581,.T.);
#9425=FACE_OUTER_BOUND('',#15582,.T.);
#9426=FACE_OUTER_BOUND('',#15583,.T.);
#9427=FACE_OUTER_BOUND('',#15584,.T.);
#9428=FACE_OUTER_BOUND('',#15585,.T.);
#9429=FACE_OUTER_BOUND('',#15586,.T.);
#9430=FACE_OUTER_BOUND('',#15587,.T.);
#9431=FACE_OUTER_BOUND('',#15588,.T.);
#9432=FACE_OUTER_BOUND('',#15589,.T.);
#9433=FACE_OUTER_BOUND('',#15590,.T.);
#9434=FACE_OUTER_BOUND('',#15591,.T.);
#9435=FACE_OUTER_BOUND('',#15592,.T.);
#9436=FACE_OUTER_BOUND('',#15593,.T.);
#9437=FACE_OUTER_BOUND('',#15594,.T.);
#9438=FACE_OUTER_BOUND('',#15595,.T.);
#9439=FACE_OUTER_BOUND('',#15596,.T.);
#9440=FACE_OUTER_BOUND('',#15597,.T.);
#9441=FACE_OUTER_BOUND('',#15598,.T.);
#9442=FACE_OUTER_BOUND('',#15599,.T.);
#9443=FACE_OUTER_BOUND('',#15600,.T.);
#9444=FACE_OUTER_BOUND('',#15601,.T.);
#9445=FACE_OUTER_BOUND('',#15602,.T.);
#9446=FACE_OUTER_BOUND('',#15603,.T.);
#9447=FACE_OUTER_BOUND('',#15604,.T.);
#9448=FACE_OUTER_BOUND('',#15605,.T.);
#9449=FACE_OUTER_BOUND('',#15606,.T.);
#9450=FACE_OUTER_BOUND('',#15607,.T.);
#9451=FACE_OUTER_BOUND('',#15608,.T.);
#9452=FACE_OUTER_BOUND('',#15609,.T.);
#9453=FACE_OUTER_BOUND('',#15610,.T.);
#9454=FACE_OUTER_BOUND('',#15611,.T.);
#9455=FACE_OUTER_BOUND('',#15612,.T.);
#9456=FACE_OUTER_BOUND('',#15613,.T.);
#9457=FACE_OUTER_BOUND('',#15614,.T.);
#9458=FACE_OUTER_BOUND('',#15615,.T.);
#9459=FACE_OUTER_BOUND('',#15616,.T.);
#9460=FACE_OUTER_BOUND('',#15617,.T.);
#9461=FACE_OUTER_BOUND('',#15618,.T.);
#9462=FACE_OUTER_BOUND('',#15619,.T.);
#9463=FACE_OUTER_BOUND('',#15620,.T.);
#9464=FACE_OUTER_BOUND('',#15621,.T.);
#9465=FACE_OUTER_BOUND('',#15622,.T.);
#9466=FACE_OUTER_BOUND('',#15623,.T.);
#9467=FACE_OUTER_BOUND('',#15624,.T.);
#9468=FACE_OUTER_BOUND('',#15625,.T.);
#9469=FACE_OUTER_BOUND('',#15626,.T.);
#9470=FACE_OUTER_BOUND('',#15627,.T.);
#9471=FACE_OUTER_BOUND('',#15628,.T.);
#9472=FACE_OUTER_BOUND('',#15629,.T.);
#9473=FACE_OUTER_BOUND('',#15630,.T.);
#9474=FACE_OUTER_BOUND('',#15631,.T.);
#9475=FACE_OUTER_BOUND('',#15632,.T.);
#9476=FACE_OUTER_BOUND('',#15633,.T.);
#9477=FACE_OUTER_BOUND('',#15634,.T.);
#9478=FACE_OUTER_BOUND('',#15635,.T.);
#9479=FACE_OUTER_BOUND('',#15636,.T.);
#9480=FACE_OUTER_BOUND('',#15637,.T.);
#9481=FACE_OUTER_BOUND('',#15638,.T.);
#9482=FACE_OUTER_BOUND('',#15639,.T.);
#9483=FACE_OUTER_BOUND('',#15640,.T.);
#9484=FACE_OUTER_BOUND('',#15641,.T.);
#9485=FACE_OUTER_BOUND('',#15642,.T.);
#9486=FACE_OUTER_BOUND('',#15643,.T.);
#9487=FACE_OUTER_BOUND('',#15644,.T.);
#9488=FACE_OUTER_BOUND('',#15645,.T.);
#9489=FACE_OUTER_BOUND('',#15646,.T.);
#9490=FACE_OUTER_BOUND('',#15647,.T.);
#9491=FACE_OUTER_BOUND('',#15648,.T.);
#9492=FACE_OUTER_BOUND('',#15649,.T.);
#9493=FACE_OUTER_BOUND('',#15650,.T.);
#9494=FACE_OUTER_BOUND('',#15651,.T.);
#9495=FACE_OUTER_BOUND('',#15652,.T.);
#9496=FACE_OUTER_BOUND('',#15653,.T.);
#9497=FACE_OUTER_BOUND('',#15654,.T.);
#9498=FACE_OUTER_BOUND('',#15655,.T.);
#9499=FACE_OUTER_BOUND('',#15656,.T.);
#9500=FACE_OUTER_BOUND('',#15657,.T.);
#9501=FACE_OUTER_BOUND('',#15658,.T.);
#9502=FACE_OUTER_BOUND('',#15659,.T.);
#9503=FACE_OUTER_BOUND('',#15660,.T.);
#9504=FACE_OUTER_BOUND('',#15661,.T.);
#9505=FACE_OUTER_BOUND('',#15662,.T.);
#9506=FACE_OUTER_BOUND('',#15663,.T.);
#9507=FACE_OUTER_BOUND('',#15664,.T.);
#9508=FACE_OUTER_BOUND('',#15665,.T.);
#9509=FACE_OUTER_BOUND('',#15666,.T.);
#9510=FACE_OUTER_BOUND('',#15667,.T.);
#9511=FACE_OUTER_BOUND('',#15668,.T.);
#9512=FACE_OUTER_BOUND('',#15669,.T.);
#9513=FACE_OUTER_BOUND('',#15670,.T.);
#9514=FACE_OUTER_BOUND('',#15671,.T.);
#9515=FACE_OUTER_BOUND('',#15672,.T.);
#9516=FACE_OUTER_BOUND('',#15673,.T.);
#9517=FACE_OUTER_BOUND('',#15674,.T.);
#9518=FACE_OUTER_BOUND('',#15675,.T.);
#9519=FACE_OUTER_BOUND('',#15676,.T.);
#9520=FACE_OUTER_BOUND('',#15677,.T.);
#9521=FACE_OUTER_BOUND('',#15678,.T.);
#9522=FACE_OUTER_BOUND('',#15679,.T.);
#9523=FACE_OUTER_BOUND('',#15680,.T.);
#9524=FACE_OUTER_BOUND('',#15681,.T.);
#9525=FACE_OUTER_BOUND('',#15682,.T.);
#9526=FACE_OUTER_BOUND('',#15683,.T.);
#9527=FACE_OUTER_BOUND('',#15684,.T.);
#9528=FACE_OUTER_BOUND('',#15685,.T.);
#9529=FACE_OUTER_BOUND('',#15686,.T.);
#9530=FACE_OUTER_BOUND('',#15687,.T.);
#9531=FACE_OUTER_BOUND('',#15688,.T.);
#9532=FACE_OUTER_BOUND('',#15689,.T.);
#9533=FACE_OUTER_BOUND('',#15690,.T.);
#9534=FACE_OUTER_BOUND('',#15691,.T.);
#9535=FACE_OUTER_BOUND('',#15692,.T.);
#9536=FACE_OUTER_BOUND('',#15693,.T.);
#9537=FACE_OUTER_BOUND('',#15694,.T.);
#9538=FACE_OUTER_BOUND('',#15695,.T.);
#9539=FACE_OUTER_BOUND('',#15696,.T.);
#9540=FACE_OUTER_BOUND('',#15697,.T.);
#9541=FACE_OUTER_BOUND('',#15698,.T.);
#9542=FACE_OUTER_BOUND('',#15699,.T.);
#9543=FACE_OUTER_BOUND('',#15700,.T.);
#9544=FACE_OUTER_BOUND('',#15701,.T.);
#9545=FACE_OUTER_BOUND('',#15702,.T.);
#9546=FACE_OUTER_BOUND('',#15703,.T.);
#9547=FACE_OUTER_BOUND('',#15704,.T.);
#9548=FACE_OUTER_BOUND('',#15705,.T.);
#9549=FACE_OUTER_BOUND('',#15706,.T.);
#9550=FACE_OUTER_BOUND('',#15707,.T.);
#9551=FACE_OUTER_BOUND('',#15708,.T.);
#9552=FACE_OUTER_BOUND('',#15709,.T.);
#9553=FACE_OUTER_BOUND('',#15710,.T.);
#9554=FACE_OUTER_BOUND('',#15711,.T.);
#9555=FACE_OUTER_BOUND('',#15712,.T.);
#9556=FACE_OUTER_BOUND('',#15713,.T.);
#9557=FACE_OUTER_BOUND('',#15714,.T.);
#9558=FACE_OUTER_BOUND('',#15715,.T.);
#9559=FACE_OUTER_BOUND('',#15716,.T.);
#9560=FACE_OUTER_BOUND('',#15717,.T.);
#9561=FACE_OUTER_BOUND('',#15718,.T.);
#9562=FACE_OUTER_BOUND('',#15719,.T.);
#9563=FACE_OUTER_BOUND('',#15720,.T.);
#9564=FACE_OUTER_BOUND('',#15721,.T.);
#9565=FACE_OUTER_BOUND('',#15722,.T.);
#9566=FACE_OUTER_BOUND('',#15723,.T.);
#9567=FACE_OUTER_BOUND('',#15724,.T.);
#9568=FACE_OUTER_BOUND('',#15725,.T.);
#9569=FACE_OUTER_BOUND('',#15726,.T.);
#9570=FACE_OUTER_BOUND('',#15727,.T.);
#9571=FACE_OUTER_BOUND('',#15728,.T.);
#9572=FACE_OUTER_BOUND('',#15729,.T.);
#9573=FACE_OUTER_BOUND('',#15730,.T.);
#9574=FACE_OUTER_BOUND('',#15731,.T.);
#9575=FACE_OUTER_BOUND('',#15732,.T.);
#9576=FACE_OUTER_BOUND('',#15733,.T.);
#9577=FACE_OUTER_BOUND('',#15734,.T.);
#9578=FACE_OUTER_BOUND('',#15735,.T.);
#9579=FACE_OUTER_BOUND('',#15736,.T.);
#9580=FACE_OUTER_BOUND('',#15737,.T.);
#9581=FACE_OUTER_BOUND('',#15738,.T.);
#9582=FACE_OUTER_BOUND('',#15739,.T.);
#9583=FACE_OUTER_BOUND('',#15740,.T.);
#9584=FACE_OUTER_BOUND('',#15741,.T.);
#9585=FACE_OUTER_BOUND('',#15742,.T.);
#9586=FACE_OUTER_BOUND('',#15743,.T.);
#9587=FACE_OUTER_BOUND('',#15744,.T.);
#9588=FACE_OUTER_BOUND('',#15745,.T.);
#9589=FACE_OUTER_BOUND('',#15746,.T.);
#9590=FACE_OUTER_BOUND('',#15747,.T.);
#9591=FACE_OUTER_BOUND('',#15748,.T.);
#9592=FACE_OUTER_BOUND('',#15749,.T.);
#9593=FACE_OUTER_BOUND('',#15750,.T.);
#9594=FACE_OUTER_BOUND('',#15751,.T.);
#9595=FACE_OUTER_BOUND('',#15752,.T.);
#9596=FACE_OUTER_BOUND('',#15753,.T.);
#9597=FACE_OUTER_BOUND('',#15754,.T.);
#9598=FACE_OUTER_BOUND('',#15755,.T.);
#9599=FACE_OUTER_BOUND('',#15756,.T.);
#9600=FACE_OUTER_BOUND('',#15757,.T.);
#9601=FACE_OUTER_BOUND('',#15758,.T.);
#9602=FACE_OUTER_BOUND('',#15759,.T.);
#9603=FACE_OUTER_BOUND('',#15760,.T.);
#9604=FACE_OUTER_BOUND('',#15761,.T.);
#9605=FACE_OUTER_BOUND('',#15762,.T.);
#9606=FACE_OUTER_BOUND('',#15763,.T.);
#9607=FACE_OUTER_BOUND('',#15764,.T.);
#9608=FACE_OUTER_BOUND('',#15765,.T.);
#9609=FACE_OUTER_BOUND('',#15766,.T.);
#9610=FACE_OUTER_BOUND('',#15767,.T.);
#9611=FACE_OUTER_BOUND('',#15768,.T.);
#9612=FACE_OUTER_BOUND('',#15769,.T.);
#9613=FACE_OUTER_BOUND('',#15770,.T.);
#9614=FACE_OUTER_BOUND('',#15771,.T.);
#9615=FACE_OUTER_BOUND('',#15772,.T.);
#9616=FACE_OUTER_BOUND('',#15773,.T.);
#9617=FACE_OUTER_BOUND('',#15774,.T.);
#9618=FACE_OUTER_BOUND('',#15775,.T.);
#9619=FACE_OUTER_BOUND('',#15776,.T.);
#9620=FACE_OUTER_BOUND('',#15777,.T.);
#9621=FACE_OUTER_BOUND('',#15778,.T.);
#9622=FACE_OUTER_BOUND('',#15779,.T.);
#9623=FACE_OUTER_BOUND('',#15780,.T.);
#9624=FACE_OUTER_BOUND('',#15781,.T.);
#9625=FACE_OUTER_BOUND('',#15782,.T.);
#9626=FACE_OUTER_BOUND('',#15783,.T.);
#9627=FACE_OUTER_BOUND('',#15784,.T.);
#9628=FACE_OUTER_BOUND('',#15785,.T.);
#9629=FACE_OUTER_BOUND('',#15786,.T.);
#9630=FACE_OUTER_BOUND('',#15787,.T.);
#9631=FACE_OUTER_BOUND('',#15788,.T.);
#9632=FACE_OUTER_BOUND('',#15789,.T.);
#9633=FACE_OUTER_BOUND('',#15790,.T.);
#9634=FACE_OUTER_BOUND('',#15791,.T.);
#9635=FACE_OUTER_BOUND('',#15792,.T.);
#9636=FACE_OUTER_BOUND('',#15793,.T.);
#9637=FACE_OUTER_BOUND('',#15794,.T.);
#9638=FACE_OUTER_BOUND('',#15795,.T.);
#9639=FACE_OUTER_BOUND('',#15796,.T.);
#9640=FACE_OUTER_BOUND('',#15797,.T.);
#9641=FACE_OUTER_BOUND('',#15798,.T.);
#9642=FACE_OUTER_BOUND('',#15799,.T.);
#9643=FACE_OUTER_BOUND('',#15800,.T.);
#9644=FACE_OUTER_BOUND('',#15801,.T.);
#9645=FACE_OUTER_BOUND('',#15802,.T.);
#9646=FACE_OUTER_BOUND('',#15803,.T.);
#9647=FACE_OUTER_BOUND('',#15804,.T.);
#9648=FACE_OUTER_BOUND('',#15805,.T.);
#9649=FACE_OUTER_BOUND('',#15806,.T.);
#9650=FACE_OUTER_BOUND('',#15807,.T.);
#9651=FACE_OUTER_BOUND('',#15808,.T.);
#9652=FACE_OUTER_BOUND('',#15809,.T.);
#9653=FACE_OUTER_BOUND('',#15810,.T.);
#9654=FACE_OUTER_BOUND('',#15811,.T.);
#9655=FACE_OUTER_BOUND('',#15812,.T.);
#9656=FACE_OUTER_BOUND('',#15813,.T.);
#9657=FACE_OUTER_BOUND('',#15814,.T.);
#9658=FACE_OUTER_BOUND('',#15815,.T.);
#9659=FACE_OUTER_BOUND('',#15816,.T.);
#9660=FACE_OUTER_BOUND('',#15817,.T.);
#9661=FACE_OUTER_BOUND('',#15818,.T.);
#9662=FACE_OUTER_BOUND('',#15819,.T.);
#9663=FACE_OUTER_BOUND('',#15820,.T.);
#9664=FACE_OUTER_BOUND('',#15821,.T.);
#9665=FACE_OUTER_BOUND('',#15822,.T.);
#9666=FACE_OUTER_BOUND('',#15823,.T.);
#9667=FACE_OUTER_BOUND('',#15824,.T.);
#9668=FACE_OUTER_BOUND('',#15825,.T.);
#9669=FACE_OUTER_BOUND('',#15826,.T.);
#9670=FACE_OUTER_BOUND('',#15827,.T.);
#9671=FACE_OUTER_BOUND('',#15828,.T.);
#9672=FACE_OUTER_BOUND('',#15829,.T.);
#9673=FACE_OUTER_BOUND('',#15830,.T.);
#9674=FACE_OUTER_BOUND('',#15831,.T.);
#9675=FACE_OUTER_BOUND('',#15832,.T.);
#9676=FACE_OUTER_BOUND('',#15833,.T.);
#9677=FACE_OUTER_BOUND('',#15834,.T.);
#9678=FACE_OUTER_BOUND('',#15835,.T.);
#9679=FACE_OUTER_BOUND('',#15836,.T.);
#9680=FACE_OUTER_BOUND('',#15837,.T.);
#9681=FACE_OUTER_BOUND('',#15838,.T.);
#9682=FACE_OUTER_BOUND('',#15839,.T.);
#9683=FACE_OUTER_BOUND('',#15840,.T.);
#9684=FACE_OUTER_BOUND('',#15841,.T.);
#9685=FACE_OUTER_BOUND('',#15842,.T.);
#9686=FACE_OUTER_BOUND('',#15843,.T.);
#9687=FACE_OUTER_BOUND('',#15844,.T.);
#9688=FACE_OUTER_BOUND('',#15845,.T.);
#9689=FACE_OUTER_BOUND('',#15846,.T.);
#9690=FACE_OUTER_BOUND('',#15847,.T.);
#9691=FACE_OUTER_BOUND('',#15848,.T.);
#9692=FACE_OUTER_BOUND('',#15849,.T.);
#9693=FACE_OUTER_BOUND('',#15850,.T.);
#9694=FACE_OUTER_BOUND('',#15851,.T.);
#9695=FACE_OUTER_BOUND('',#15852,.T.);
#9696=FACE_OUTER_BOUND('',#15853,.T.);
#9697=FACE_OUTER_BOUND('',#15854,.T.);
#9698=FACE_OUTER_BOUND('',#15855,.T.);
#9699=FACE_OUTER_BOUND('',#15856,.T.);
#9700=FACE_OUTER_BOUND('',#15857,.T.);
#9701=FACE_OUTER_BOUND('',#15858,.T.);
#9702=FACE_OUTER_BOUND('',#15859,.T.);
#9703=FACE_OUTER_BOUND('',#15860,.T.);
#9704=FACE_OUTER_BOUND('',#15861,.T.);
#9705=FACE_OUTER_BOUND('',#15862,.T.);
#9706=FACE_OUTER_BOUND('',#15863,.T.);
#9707=FACE_OUTER_BOUND('',#15864,.T.);
#9708=FACE_OUTER_BOUND('',#15865,.T.);
#9709=FACE_OUTER_BOUND('',#15866,.T.);
#9710=FACE_OUTER_BOUND('',#15867,.T.);
#9711=FACE_OUTER_BOUND('',#15868,.T.);
#9712=FACE_OUTER_BOUND('',#15869,.T.);
#9713=FACE_OUTER_BOUND('',#15870,.T.);
#9714=FACE_OUTER_BOUND('',#15871,.T.);
#9715=FACE_OUTER_BOUND('',#15872,.T.);
#9716=FACE_OUTER_BOUND('',#15873,.T.);
#9717=FACE_OUTER_BOUND('',#15874,.T.);
#9718=FACE_OUTER_BOUND('',#15875,.T.);
#9719=FACE_OUTER_BOUND('',#15876,.T.);
#9720=FACE_OUTER_BOUND('',#15877,.T.);
#9721=FACE_OUTER_BOUND('',#15878,.T.);
#9722=FACE_OUTER_BOUND('',#15879,.T.);
#9723=FACE_OUTER_BOUND('',#15880,.T.);
#9724=FACE_OUTER_BOUND('',#15881,.T.);
#9725=FACE_OUTER_BOUND('',#15882,.T.);
#9726=FACE_OUTER_BOUND('',#15883,.T.);
#9727=FACE_OUTER_BOUND('',#15884,.T.);
#9728=FACE_OUTER_BOUND('',#15885,.T.);
#9729=FACE_OUTER_BOUND('',#15886,.T.);
#9730=FACE_OUTER_BOUND('',#15887,.T.);
#9731=FACE_OUTER_BOUND('',#15888,.T.);
#9732=FACE_OUTER_BOUND('',#15889,.T.);
#9733=FACE_OUTER_BOUND('',#15890,.T.);
#9734=FACE_OUTER_BOUND('',#15891,.T.);
#9735=FACE_OUTER_BOUND('',#15892,.T.);
#9736=FACE_OUTER_BOUND('',#15893,.T.);
#9737=FACE_OUTER_BOUND('',#15894,.T.);
#9738=FACE_OUTER_BOUND('',#15895,.T.);
#9739=FACE_OUTER_BOUND('',#15896,.T.);
#9740=FACE_OUTER_BOUND('',#15897,.T.);
#9741=FACE_OUTER_BOUND('',#15898,.T.);
#9742=FACE_OUTER_BOUND('',#15899,.T.);
#9743=FACE_OUTER_BOUND('',#15900,.T.);
#9744=FACE_OUTER_BOUND('',#15901,.T.);
#9745=FACE_OUTER_BOUND('',#15902,.T.);
#9746=FACE_OUTER_BOUND('',#15903,.T.);
#9747=FACE_OUTER_BOUND('',#15904,.T.);
#9748=FACE_OUTER_BOUND('',#15905,.T.);
#9749=FACE_OUTER_BOUND('',#15906,.T.);
#9750=FACE_OUTER_BOUND('',#15907,.T.);
#9751=FACE_OUTER_BOUND('',#15908,.T.);
#9752=FACE_OUTER_BOUND('',#15909,.T.);
#9753=FACE_OUTER_BOUND('',#15910,.T.);
#9754=FACE_OUTER_BOUND('',#15911,.T.);
#9755=FACE_OUTER_BOUND('',#15912,.T.);
#9756=FACE_OUTER_BOUND('',#15913,.T.);
#9757=FACE_OUTER_BOUND('',#15914,.T.);
#9758=FACE_OUTER_BOUND('',#15915,.T.);
#9759=FACE_OUTER_BOUND('',#15916,.T.);
#9760=FACE_OUTER_BOUND('',#15917,.T.);
#9761=FACE_OUTER_BOUND('',#15918,.T.);
#9762=FACE_OUTER_BOUND('',#15919,.T.);
#9763=FACE_OUTER_BOUND('',#15920,.T.);
#9764=FACE_OUTER_BOUND('',#15921,.T.);
#9765=FACE_OUTER_BOUND('',#15922,.T.);
#9766=FACE_OUTER_BOUND('',#15923,.T.);
#9767=FACE_OUTER_BOUND('',#15924,.T.);
#9768=FACE_OUTER_BOUND('',#15925,.T.);
#9769=FACE_OUTER_BOUND('',#15926,.T.);
#9770=FACE_OUTER_BOUND('',#15927,.T.);
#9771=FACE_OUTER_BOUND('',#15928,.T.);
#9772=FACE_OUTER_BOUND('',#15929,.T.);
#9773=FACE_OUTER_BOUND('',#15930,.T.);
#9774=FACE_OUTER_BOUND('',#15931,.T.);
#9775=FACE_OUTER_BOUND('',#15932,.T.);
#9776=FACE_OUTER_BOUND('',#15933,.T.);
#9777=FACE_OUTER_BOUND('',#15934,.T.);
#9778=FACE_OUTER_BOUND('',#15935,.T.);
#9779=FACE_OUTER_BOUND('',#15936,.T.);
#9780=FACE_OUTER_BOUND('',#15937,.T.);
#9781=FACE_OUTER_BOUND('',#15938,.T.);
#9782=FACE_OUTER_BOUND('',#15939,.T.);
#9783=FACE_OUTER_BOUND('',#15940,.T.);
#9784=FACE_OUTER_BOUND('',#15941,.T.);
#9785=FACE_OUTER_BOUND('',#15942,.T.);
#9786=FACE_OUTER_BOUND('',#15943,.T.);
#9787=FACE_OUTER_BOUND('',#15944,.T.);
#9788=FACE_OUTER_BOUND('',#15945,.T.);
#9789=FACE_OUTER_BOUND('',#15946,.T.);
#9790=FACE_OUTER_BOUND('',#15947,.T.);
#9791=FACE_OUTER_BOUND('',#15948,.T.);
#9792=FACE_OUTER_BOUND('',#15949,.T.);
#9793=FACE_OUTER_BOUND('',#15950,.T.);
#9794=FACE_OUTER_BOUND('',#15951,.T.);
#9795=FACE_OUTER_BOUND('',#15952,.T.);
#9796=FACE_OUTER_BOUND('',#15953,.T.);
#9797=FACE_OUTER_BOUND('',#15954,.T.);
#9798=FACE_OUTER_BOUND('',#15955,.T.);
#9799=FACE_OUTER_BOUND('',#15956,.T.);
#9800=FACE_OUTER_BOUND('',#15957,.T.);
#9801=FACE_OUTER_BOUND('',#15958,.T.);
#9802=FACE_OUTER_BOUND('',#15959,.T.);
#9803=FACE_OUTER_BOUND('',#15960,.T.);
#9804=FACE_OUTER_BOUND('',#15961,.T.);
#9805=FACE_OUTER_BOUND('',#15962,.T.);
#9806=FACE_OUTER_BOUND('',#15963,.T.);
#9807=FACE_OUTER_BOUND('',#15964,.T.);
#9808=FACE_OUTER_BOUND('',#15965,.T.);
#9809=FACE_OUTER_BOUND('',#15966,.T.);
#9810=FACE_OUTER_BOUND('',#15967,.T.);
#9811=FACE_OUTER_BOUND('',#15968,.T.);
#9812=FACE_OUTER_BOUND('',#15969,.T.);
#9813=FACE_OUTER_BOUND('',#15970,.T.);
#9814=FACE_OUTER_BOUND('',#15971,.T.);
#9815=FACE_OUTER_BOUND('',#15972,.T.);
#9816=FACE_OUTER_BOUND('',#15973,.T.);
#9817=FACE_OUTER_BOUND('',#15974,.T.);
#9818=FACE_OUTER_BOUND('',#15975,.T.);
#9819=FACE_OUTER_BOUND('',#15976,.T.);
#9820=FACE_OUTER_BOUND('',#15977,.T.);
#9821=FACE_OUTER_BOUND('',#15978,.T.);
#9822=FACE_OUTER_BOUND('',#15979,.T.);
#9823=FACE_OUTER_BOUND('',#15980,.T.);
#9824=FACE_OUTER_BOUND('',#15981,.T.);
#9825=FACE_OUTER_BOUND('',#15982,.T.);
#9826=FACE_OUTER_BOUND('',#15983,.T.);
#9827=FACE_OUTER_BOUND('',#15984,.T.);
#9828=FACE_OUTER_BOUND('',#15985,.T.);
#9829=FACE_OUTER_BOUND('',#15986,.T.);
#9830=FACE_OUTER_BOUND('',#15987,.T.);
#9831=FACE_OUTER_BOUND('',#15988,.T.);
#9832=FACE_OUTER_BOUND('',#15989,.T.);
#9833=FACE_OUTER_BOUND('',#15990,.T.);
#9834=FACE_OUTER_BOUND('',#15991,.T.);
#9835=FACE_OUTER_BOUND('',#15992,.T.);
#9836=FACE_OUTER_BOUND('',#15993,.T.);
#9837=FACE_OUTER_BOUND('',#15994,.T.);
#9838=FACE_OUTER_BOUND('',#15995,.T.);
#9839=FACE_OUTER_BOUND('',#15996,.T.);
#9840=FACE_OUTER_BOUND('',#15997,.T.);
#9841=FACE_OUTER_BOUND('',#15998,.T.);
#9842=FACE_OUTER_BOUND('',#15999,.T.);
#9843=FACE_OUTER_BOUND('',#16000,.T.);
#9844=FACE_OUTER_BOUND('',#16001,.T.);
#9845=FACE_OUTER_BOUND('',#16002,.T.);
#9846=FACE_OUTER_BOUND('',#16003,.T.);
#9847=FACE_OUTER_BOUND('',#16004,.T.);
#9848=FACE_OUTER_BOUND('',#16005,.T.);
#9849=FACE_OUTER_BOUND('',#16006,.T.);
#9850=FACE_OUTER_BOUND('',#16007,.T.);
#9851=FACE_OUTER_BOUND('',#16008,.T.);
#9852=FACE_OUTER_BOUND('',#16009,.T.);
#9853=FACE_OUTER_BOUND('',#16010,.T.);
#9854=FACE_OUTER_BOUND('',#16011,.T.);
#9855=FACE_OUTER_BOUND('',#16012,.T.);
#9856=FACE_OUTER_BOUND('',#16013,.T.);
#9857=FACE_OUTER_BOUND('',#16014,.T.);
#9858=FACE_OUTER_BOUND('',#16015,.T.);
#9859=FACE_OUTER_BOUND('',#16016,.T.);
#9860=FACE_OUTER_BOUND('',#16017,.T.);
#9861=FACE_OUTER_BOUND('',#16018,.T.);
#9862=FACE_OUTER_BOUND('',#16019,.T.);
#9863=FACE_OUTER_BOUND('',#16020,.T.);
#9864=FACE_OUTER_BOUND('',#16021,.T.);
#9865=FACE_OUTER_BOUND('',#16022,.T.);
#9866=FACE_OUTER_BOUND('',#16023,.T.);
#9867=FACE_OUTER_BOUND('',#16024,.T.);
#9868=FACE_OUTER_BOUND('',#16025,.T.);
#9869=FACE_OUTER_BOUND('',#16026,.T.);
#9870=FACE_OUTER_BOUND('',#16027,.T.);
#9871=FACE_OUTER_BOUND('',#16028,.T.);
#9872=FACE_OUTER_BOUND('',#16029,.T.);
#9873=FACE_OUTER_BOUND('',#16030,.T.);
#9874=FACE_OUTER_BOUND('',#16031,.T.);
#9875=FACE_OUTER_BOUND('',#16032,.T.);
#9876=FACE_OUTER_BOUND('',#16033,.T.);
#9877=FACE_OUTER_BOUND('',#16034,.T.);
#9878=FACE_OUTER_BOUND('',#16035,.T.);
#9879=FACE_OUTER_BOUND('',#16036,.T.);
#9880=FACE_OUTER_BOUND('',#16037,.T.);
#9881=FACE_OUTER_BOUND('',#16038,.T.);
#9882=FACE_OUTER_BOUND('',#16039,.T.);
#9883=FACE_OUTER_BOUND('',#16040,.T.);
#9884=FACE_OUTER_BOUND('',#16041,.T.);
#9885=FACE_OUTER_BOUND('',#16042,.T.);
#9886=FACE_OUTER_BOUND('',#16043,.T.);
#9887=FACE_OUTER_BOUND('',#16044,.T.);
#9888=FACE_OUTER_BOUND('',#16045,.T.);
#9889=FACE_OUTER_BOUND('',#16046,.T.);
#9890=FACE_OUTER_BOUND('',#16047,.T.);
#9891=FACE_OUTER_BOUND('',#16048,.T.);
#9892=FACE_OUTER_BOUND('',#16049,.T.);
#9893=FACE_OUTER_BOUND('',#16050,.T.);
#9894=FACE_OUTER_BOUND('',#16051,.T.);
#9895=FACE_OUTER_BOUND('',#16052,.T.);
#9896=FACE_OUTER_BOUND('',#16053,.T.);
#9897=FACE_OUTER_BOUND('',#16054,.T.);
#9898=FACE_OUTER_BOUND('',#16055,.T.);
#9899=FACE_OUTER_BOUND('',#16056,.T.);
#9900=FACE_OUTER_BOUND('',#16057,.T.);
#9901=FACE_OUTER_BOUND('',#16058,.T.);
#9902=FACE_OUTER_BOUND('',#16059,.T.);
#9903=FACE_OUTER_BOUND('',#16060,.T.);
#9904=FACE_OUTER_BOUND('',#16061,.T.);
#9905=FACE_OUTER_BOUND('',#16062,.T.);
#9906=FACE_OUTER_BOUND('',#16063,.T.);
#9907=FACE_OUTER_BOUND('',#16064,.T.);
#9908=FACE_OUTER_BOUND('',#16065,.T.);
#9909=FACE_OUTER_BOUND('',#16066,.T.);
#9910=FACE_OUTER_BOUND('',#16067,.T.);
#9911=FACE_OUTER_BOUND('',#16068,.T.);
#9912=FACE_OUTER_BOUND('',#16069,.T.);
#9913=FACE_OUTER_BOUND('',#16070,.T.);
#9914=FACE_OUTER_BOUND('',#16071,.T.);
#9915=FACE_OUTER_BOUND('',#16072,.T.);
#9916=FACE_OUTER_BOUND('',#16073,.T.);
#9917=FACE_OUTER_BOUND('',#16074,.T.);
#9918=FACE_OUTER_BOUND('',#16075,.T.);
#9919=FACE_OUTER_BOUND('',#16076,.T.);
#9920=FACE_OUTER_BOUND('',#16077,.T.);
#9921=FACE_OUTER_BOUND('',#16078,.T.);
#9922=FACE_OUTER_BOUND('',#16079,.T.);
#9923=FACE_OUTER_BOUND('',#16080,.T.);
#9924=FACE_OUTER_BOUND('',#16081,.T.);
#9925=FACE_OUTER_BOUND('',#16082,.T.);
#9926=FACE_OUTER_BOUND('',#16083,.T.);
#9927=FACE_OUTER_BOUND('',#16084,.T.);
#9928=FACE_OUTER_BOUND('',#16085,.T.);
#9929=FACE_OUTER_BOUND('',#16086,.T.);
#9930=FACE_OUTER_BOUND('',#16087,.T.);
#9931=FACE_OUTER_BOUND('',#16088,.T.);
#9932=FACE_OUTER_BOUND('',#16089,.T.);
#9933=FACE_OUTER_BOUND('',#16090,.T.);
#9934=FACE_OUTER_BOUND('',#16091,.T.);
#9935=FACE_OUTER_BOUND('',#16092,.T.);
#9936=FACE_OUTER_BOUND('',#16093,.T.);
#9937=FACE_OUTER_BOUND('',#16094,.T.);
#9938=FACE_OUTER_BOUND('',#16095,.T.);
#9939=FACE_OUTER_BOUND('',#16096,.T.);
#9940=FACE_OUTER_BOUND('',#16097,.T.);
#9941=FACE_OUTER_BOUND('',#16098,.T.);
#9942=FACE_OUTER_BOUND('',#16099,.T.);
#9943=FACE_OUTER_BOUND('',#16100,.T.);
#9944=FACE_OUTER_BOUND('',#16101,.T.);
#9945=FACE_OUTER_BOUND('',#16102,.T.);
#9946=FACE_OUTER_BOUND('',#16103,.T.);
#9947=FACE_OUTER_BOUND('',#16104,.T.);
#9948=FACE_OUTER_BOUND('',#16105,.T.);
#9949=FACE_OUTER_BOUND('',#16106,.T.);
#9950=FACE_OUTER_BOUND('',#16107,.T.);
#9951=FACE_OUTER_BOUND('',#16108,.T.);
#9952=FACE_OUTER_BOUND('',#16109,.T.);
#9953=FACE_OUTER_BOUND('',#16110,.T.);
#9954=FACE_OUTER_BOUND('',#16111,.T.);
#9955=FACE_OUTER_BOUND('',#16112,.T.);
#9956=FACE_OUTER_BOUND('',#16113,.T.);
#9957=FACE_OUTER_BOUND('',#16114,.T.);
#9958=FACE_OUTER_BOUND('',#16115,.T.);
#9959=FACE_OUTER_BOUND('',#16116,.T.);
#9960=FACE_OUTER_BOUND('',#16117,.T.);
#9961=FACE_OUTER_BOUND('',#16118,.T.);
#9962=FACE_OUTER_BOUND('',#16119,.T.);
#9963=FACE_OUTER_BOUND('',#16120,.T.);
#9964=FACE_OUTER_BOUND('',#16121,.T.);
#9965=FACE_OUTER_BOUND('',#16122,.T.);
#9966=FACE_OUTER_BOUND('',#16123,.T.);
#9967=FACE_OUTER_BOUND('',#16124,.T.);
#9968=FACE_OUTER_BOUND('',#16125,.T.);
#9969=FACE_OUTER_BOUND('',#16126,.T.);
#9970=FACE_OUTER_BOUND('',#16127,.T.);
#9971=FACE_OUTER_BOUND('',#16128,.T.);
#9972=FACE_OUTER_BOUND('',#16129,.T.);
#9973=FACE_OUTER_BOUND('',#16130,.T.);
#9974=FACE_OUTER_BOUND('',#16131,.T.);
#9975=FACE_OUTER_BOUND('',#16132,.T.);
#9976=FACE_OUTER_BOUND('',#16133,.T.);
#9977=FACE_OUTER_BOUND('',#16134,.T.);
#9978=FACE_OUTER_BOUND('',#16135,.T.);
#9979=FACE_OUTER_BOUND('',#16136,.T.);
#9980=FACE_OUTER_BOUND('',#16137,.T.);
#9981=FACE_OUTER_BOUND('',#16138,.T.);
#9982=FACE_OUTER_BOUND('',#16139,.T.);
#9983=FACE_OUTER_BOUND('',#16140,.T.);
#9984=FACE_OUTER_BOUND('',#16141,.T.);
#9985=FACE_OUTER_BOUND('',#16142,.T.);
#9986=FACE_OUTER_BOUND('',#16143,.T.);
#9987=FACE_OUTER_BOUND('',#16144,.T.);
#9988=FACE_OUTER_BOUND('',#16145,.T.);
#9989=FACE_OUTER_BOUND('',#16146,.T.);
#9990=FACE_OUTER_BOUND('',#16147,.T.);
#9991=FACE_OUTER_BOUND('',#16148,.T.);
#9992=FACE_OUTER_BOUND('',#16149,.T.);
#9993=FACE_OUTER_BOUND('',#16150,.T.);
#9994=FACE_OUTER_BOUND('',#16151,.T.);
#9995=FACE_OUTER_BOUND('',#16152,.T.);
#9996=FACE_OUTER_BOUND('',#16153,.T.);
#9997=FACE_OUTER_BOUND('',#16154,.T.);
#9998=FACE_OUTER_BOUND('',#16155,.T.);
#9999=FACE_OUTER_BOUND('',#16156,.T.);
#10000=FACE_OUTER_BOUND('',#16157,.T.);
#10001=FACE_OUTER_BOUND('',#16158,.T.);
#10002=FACE_OUTER_BOUND('',#16159,.T.);
#10003=FACE_OUTER_BOUND('',#16160,.T.);
#10004=FACE_OUTER_BOUND('',#16161,.T.);
#10005=FACE_OUTER_BOUND('',#16162,.T.);
#10006=FACE_OUTER_BOUND('',#16163,.T.);
#10007=FACE_OUTER_BOUND('',#16164,.T.);
#10008=FACE_OUTER_BOUND('',#16165,.T.);
#10009=FACE_OUTER_BOUND('',#16166,.T.);
#10010=FACE_OUTER_BOUND('',#16167,.T.);
#10011=FACE_OUTER_BOUND('',#16168,.T.);
#10012=FACE_OUTER_BOUND('',#16169,.T.);
#10013=FACE_OUTER_BOUND('',#16170,.T.);
#10014=FACE_OUTER_BOUND('',#16171,.T.);
#10015=FACE_OUTER_BOUND('',#16172,.T.);
#10016=FACE_OUTER_BOUND('',#16173,.T.);
#10017=FACE_OUTER_BOUND('',#16174,.T.);
#10018=FACE_OUTER_BOUND('',#16175,.T.);
#10019=FACE_OUTER_BOUND('',#16176,.T.);
#10020=FACE_OUTER_BOUND('',#16177,.T.);
#10021=FACE_OUTER_BOUND('',#16178,.T.);
#10022=FACE_OUTER_BOUND('',#16179,.T.);
#10023=FACE_OUTER_BOUND('',#16180,.T.);
#10024=FACE_OUTER_BOUND('',#16181,.T.);
#10025=FACE_OUTER_BOUND('',#16182,.T.);
#10026=FACE_OUTER_BOUND('',#16183,.T.);
#10027=FACE_OUTER_BOUND('',#16184,.T.);
#10028=FACE_OUTER_BOUND('',#16185,.T.);
#10029=FACE_OUTER_BOUND('',#16186,.T.);
#10030=FACE_OUTER_BOUND('',#16187,.T.);
#10031=FACE_OUTER_BOUND('',#16188,.T.);
#10032=FACE_OUTER_BOUND('',#16189,.T.);
#10033=FACE_OUTER_BOUND('',#16190,.T.);
#10034=FACE_OUTER_BOUND('',#16191,.T.);
#10035=FACE_OUTER_BOUND('',#16192,.T.);
#10036=FACE_OUTER_BOUND('',#16193,.T.);
#10037=FACE_OUTER_BOUND('',#16194,.T.);
#10038=FACE_OUTER_BOUND('',#16195,.T.);
#10039=FACE_OUTER_BOUND('',#16196,.T.);
#10040=FACE_OUTER_BOUND('',#16197,.T.);
#10041=FACE_OUTER_BOUND('',#16198,.T.);
#10042=FACE_OUTER_BOUND('',#16199,.T.);
#10043=FACE_OUTER_BOUND('',#16200,.T.);
#10044=FACE_OUTER_BOUND('',#16201,.T.);
#10045=FACE_OUTER_BOUND('',#16202,.T.);
#10046=FACE_OUTER_BOUND('',#16203,.T.);
#10047=FACE_OUTER_BOUND('',#16204,.T.);
#10048=FACE_OUTER_BOUND('',#16205,.T.);
#10049=FACE_OUTER_BOUND('',#16206,.T.);
#10050=FACE_OUTER_BOUND('',#16207,.T.);
#10051=FACE_OUTER_BOUND('',#16208,.T.);
#10052=FACE_OUTER_BOUND('',#16209,.T.);
#10053=FACE_OUTER_BOUND('',#16210,.T.);
#10054=FACE_OUTER_BOUND('',#16211,.T.);
#10055=FACE_OUTER_BOUND('',#16212,.T.);
#10056=FACE_OUTER_BOUND('',#16213,.T.);
#10057=FACE_OUTER_BOUND('',#16214,.T.);
#10058=FACE_OUTER_BOUND('',#16215,.T.);
#10059=FACE_OUTER_BOUND('',#16216,.T.);
#10060=FACE_OUTER_BOUND('',#16217,.T.);
#10061=FACE_OUTER_BOUND('',#16218,.T.);
#10062=FACE_OUTER_BOUND('',#16219,.T.);
#10063=FACE_OUTER_BOUND('',#16220,.T.);
#10064=FACE_OUTER_BOUND('',#16221,.T.);
#10065=FACE_OUTER_BOUND('',#16222,.T.);
#10066=FACE_OUTER_BOUND('',#16223,.T.);
#10067=FACE_OUTER_BOUND('',#16224,.T.);
#10068=FACE_OUTER_BOUND('',#16225,.T.);
#10069=FACE_OUTER_BOUND('',#16226,.T.);
#10070=FACE_OUTER_BOUND('',#16227,.T.);
#10071=FACE_OUTER_BOUND('',#16228,.T.);
#10072=FACE_OUTER_BOUND('',#16229,.T.);
#10073=FACE_OUTER_BOUND('',#16230,.T.);
#10074=FACE_OUTER_BOUND('',#16231,.T.);
#10075=FACE_OUTER_BOUND('',#16232,.T.);
#10076=FACE_OUTER_BOUND('',#16233,.T.);
#10077=FACE_OUTER_BOUND('',#16234,.T.);
#10078=FACE_OUTER_BOUND('',#16235,.T.);
#10079=FACE_OUTER_BOUND('',#16236,.T.);
#10080=FACE_OUTER_BOUND('',#16237,.T.);
#10081=FACE_OUTER_BOUND('',#16238,.T.);
#10082=FACE_OUTER_BOUND('',#16239,.T.);
#10083=FACE_OUTER_BOUND('',#16240,.T.);
#10084=FACE_OUTER_BOUND('',#16241,.T.);
#10085=FACE_OUTER_BOUND('',#16242,.T.);
#10086=FACE_OUTER_BOUND('',#16243,.T.);
#10087=FACE_OUTER_BOUND('',#16244,.T.);
#10088=FACE_OUTER_BOUND('',#16245,.T.);
#10089=FACE_OUTER_BOUND('',#16246,.T.);
#10090=FACE_OUTER_BOUND('',#16247,.T.);
#10091=FACE_OUTER_BOUND('',#16248,.T.);
#10092=FACE_OUTER_BOUND('',#16249,.T.);
#10093=FACE_OUTER_BOUND('',#16250,.T.);
#10094=FACE_OUTER_BOUND('',#16251,.T.);
#10095=FACE_OUTER_BOUND('',#16252,.T.);
#10096=FACE_OUTER_BOUND('',#16253,.T.);
#10097=FACE_OUTER_BOUND('',#16254,.T.);
#10098=FACE_OUTER_BOUND('',#16255,.T.);
#10099=FACE_OUTER_BOUND('',#16256,.T.);
#10100=FACE_OUTER_BOUND('',#16257,.T.);
#10101=FACE_OUTER_BOUND('',#16258,.T.);
#10102=FACE_OUTER_BOUND('',#16259,.T.);
#10103=FACE_OUTER_BOUND('',#16260,.T.);
#10104=FACE_OUTER_BOUND('',#16261,.T.);
#10105=FACE_OUTER_BOUND('',#16262,.T.);
#10106=FACE_OUTER_BOUND('',#16263,.T.);
#10107=FACE_OUTER_BOUND('',#16264,.T.);
#10108=FACE_OUTER_BOUND('',#16265,.T.);
#10109=FACE_OUTER_BOUND('',#16266,.T.);
#10110=FACE_OUTER_BOUND('',#16267,.T.);
#10111=FACE_OUTER_BOUND('',#16268,.T.);
#10112=FACE_OUTER_BOUND('',#16269,.T.);
#10113=FACE_OUTER_BOUND('',#16270,.T.);
#10114=FACE_OUTER_BOUND('',#16271,.T.);
#10115=FACE_OUTER_BOUND('',#16272,.T.);
#10116=FACE_OUTER_BOUND('',#16273,.T.);
#10117=FACE_OUTER_BOUND('',#16274,.T.);
#10118=FACE_OUTER_BOUND('',#16275,.T.);
#10119=FACE_OUTER_BOUND('',#16276,.T.);
#10120=FACE_OUTER_BOUND('',#16277,.T.);
#10121=FACE_OUTER_BOUND('',#16278,.T.);
#10122=FACE_OUTER_BOUND('',#16279,.T.);
#10123=FACE_OUTER_BOUND('',#16280,.T.);
#10124=FACE_OUTER_BOUND('',#16281,.T.);
#10125=FACE_OUTER_BOUND('',#16282,.T.);
#10126=FACE_OUTER_BOUND('',#16283,.T.);
#10127=FACE_OUTER_BOUND('',#16284,.T.);
#10128=FACE_OUTER_BOUND('',#16285,.T.);
#10129=FACE_OUTER_BOUND('',#16286,.T.);
#10130=FACE_OUTER_BOUND('',#16287,.T.);
#10131=FACE_OUTER_BOUND('',#16288,.T.);
#10132=FACE_OUTER_BOUND('',#16289,.T.);
#10133=FACE_OUTER_BOUND('',#16290,.T.);
#10134=FACE_OUTER_BOUND('',#16291,.T.);
#10135=FACE_OUTER_BOUND('',#16292,.T.);
#10136=FACE_OUTER_BOUND('',#16293,.T.);
#10137=FACE_OUTER_BOUND('',#16294,.T.);
#10138=FACE_OUTER_BOUND('',#16295,.T.);
#10139=FACE_OUTER_BOUND('',#16296,.T.);
#10140=FACE_OUTER_BOUND('',#16297,.T.);
#10141=FACE_OUTER_BOUND('',#16298,.T.);
#10142=FACE_OUTER_BOUND('',#16299,.T.);
#10143=FACE_OUTER_BOUND('',#16300,.T.);
#10144=FACE_OUTER_BOUND('',#16301,.T.);
#10145=FACE_OUTER_BOUND('',#16302,.T.);
#10146=FACE_OUTER_BOUND('',#16303,.T.);
#10147=FACE_OUTER_BOUND('',#16304,.T.);
#10148=FACE_OUTER_BOUND('',#16305,.T.);
#10149=FACE_OUTER_BOUND('',#16306,.T.);
#10150=FACE_OUTER_BOUND('',#16307,.T.);
#10151=FACE_OUTER_BOUND('',#16308,.T.);
#10152=FACE_OUTER_BOUND('',#16309,.T.);
#10153=FACE_OUTER_BOUND('',#16310,.T.);
#10154=FACE_OUTER_BOUND('',#16311,.T.);
#10155=FACE_OUTER_BOUND('',#16312,.T.);
#10156=FACE_OUTER_BOUND('',#16313,.T.);
#10157=FACE_OUTER_BOUND('',#16314,.T.);
#10158=FACE_OUTER_BOUND('',#16315,.T.);
#10159=FACE_OUTER_BOUND('',#16316,.T.);
#10160=FACE_OUTER_BOUND('',#16317,.T.);
#10161=FACE_OUTER_BOUND('',#16318,.T.);
#10162=FACE_OUTER_BOUND('',#16319,.T.);
#10163=FACE_OUTER_BOUND('',#16320,.T.);
#10164=FACE_OUTER_BOUND('',#16321,.T.);
#10165=FACE_OUTER_BOUND('',#16322,.T.);
#10166=FACE_OUTER_BOUND('',#16323,.T.);
#10167=FACE_OUTER_BOUND('',#16324,.T.);
#10168=FACE_OUTER_BOUND('',#16325,.T.);
#10169=FACE_OUTER_BOUND('',#16326,.T.);
#10170=FACE_OUTER_BOUND('',#16327,.T.);
#10171=FACE_OUTER_BOUND('',#16328,.T.);
#10172=FACE_OUTER_BOUND('',#16329,.T.);
#10173=FACE_OUTER_BOUND('',#16330,.T.);
#10174=FACE_OUTER_BOUND('',#16331,.T.);
#10175=FACE_OUTER_BOUND('',#16332,.T.);
#10176=FACE_OUTER_BOUND('',#16333,.T.);
#10177=FACE_OUTER_BOUND('',#16334,.T.);
#10178=FACE_OUTER_BOUND('',#16335,.T.);
#10179=FACE_OUTER_BOUND('',#16336,.T.);
#10180=FACE_OUTER_BOUND('',#16337,.T.);
#10181=FACE_OUTER_BOUND('',#16338,.T.);
#10182=FACE_OUTER_BOUND('',#16339,.T.);
#10183=FACE_OUTER_BOUND('',#16340,.T.);
#10184=FACE_OUTER_BOUND('',#16341,.T.);
#10185=FACE_OUTER_BOUND('',#16342,.T.);
#10186=FACE_OUTER_BOUND('',#16343,.T.);
#10187=FACE_OUTER_BOUND('',#16344,.T.);
#10188=FACE_OUTER_BOUND('',#16345,.T.);
#10189=FACE_OUTER_BOUND('',#16346,.T.);
#10190=FACE_OUTER_BOUND('',#16347,.T.);
#10191=FACE_OUTER_BOUND('',#16348,.T.);
#10192=FACE_OUTER_BOUND('',#16349,.T.);
#10193=FACE_OUTER_BOUND('',#16350,.T.);
#10194=FACE_OUTER_BOUND('',#16351,.T.);
#10195=FACE_OUTER_BOUND('',#16352,.T.);
#10196=FACE_OUTER_BOUND('',#16353,.T.);
#10197=FACE_OUTER_BOUND('',#16354,.T.);
#10198=FACE_OUTER_BOUND('',#16355,.T.);
#10199=FACE_OUTER_BOUND('',#16356,.T.);
#10200=FACE_OUTER_BOUND('',#16357,.T.);
#10201=FACE_OUTER_BOUND('',#16358,.T.);
#10202=FACE_OUTER_BOUND('',#16359,.T.);
#10203=FACE_OUTER_BOUND('',#16360,.T.);
#10204=FACE_OUTER_BOUND('',#16361,.T.);
#10205=FACE_OUTER_BOUND('',#16362,.T.);
#10206=FACE_OUTER_BOUND('',#16363,.T.);
#10207=FACE_OUTER_BOUND('',#16364,.T.);
#10208=FACE_OUTER_BOUND('',#16365,.T.);
#10209=FACE_OUTER_BOUND('',#16366,.T.);
#10210=FACE_OUTER_BOUND('',#16367,.T.);
#10211=FACE_OUTER_BOUND('',#16368,.T.);
#10212=FACE_OUTER_BOUND('',#16369,.T.);
#10213=FACE_OUTER_BOUND('',#16370,.T.);
#10214=FACE_OUTER_BOUND('',#16371,.T.);
#10215=FACE_OUTER_BOUND('',#16372,.T.);
#10216=FACE_OUTER_BOUND('',#16373,.T.);
#10217=FACE_OUTER_BOUND('',#16374,.T.);
#10218=FACE_OUTER_BOUND('',#16375,.T.);
#10219=FACE_OUTER_BOUND('',#16376,.T.);
#10220=FACE_OUTER_BOUND('',#16377,.T.);
#10221=FACE_OUTER_BOUND('',#16378,.T.);
#10222=FACE_OUTER_BOUND('',#16379,.T.);
#10223=FACE_OUTER_BOUND('',#16380,.T.);
#10224=FACE_OUTER_BOUND('',#16381,.T.);
#10225=FACE_OUTER_BOUND('',#16382,.T.);
#10226=FACE_OUTER_BOUND('',#16383,.T.);
#10227=FACE_OUTER_BOUND('',#16384,.T.);
#10228=FACE_OUTER_BOUND('',#16385,.T.);
#10229=FACE_OUTER_BOUND('',#16386,.T.);
#10230=FACE_OUTER_BOUND('',#16387,.T.);
#10231=FACE_OUTER_BOUND('',#16388,.T.);
#10232=FACE_OUTER_BOUND('',#16389,.T.);
#10233=FACE_OUTER_BOUND('',#16390,.T.);
#10234=FACE_OUTER_BOUND('',#16391,.T.);
#10235=FACE_OUTER_BOUND('',#16392,.T.);
#10236=FACE_OUTER_BOUND('',#16393,.T.);
#10237=FACE_OUTER_BOUND('',#16394,.T.);
#10238=FACE_OUTER_BOUND('',#16395,.T.);
#10239=FACE_OUTER_BOUND('',#16396,.T.);
#10240=FACE_OUTER_BOUND('',#16397,.T.);
#10241=FACE_OUTER_BOUND('',#16398,.T.);
#10242=FACE_OUTER_BOUND('',#16399,.T.);
#10243=FACE_OUTER_BOUND('',#16400,.T.);
#10244=FACE_OUTER_BOUND('',#16401,.T.);
#10245=FACE_OUTER_BOUND('',#16402,.T.);
#10246=FACE_OUTER_BOUND('',#16403,.T.);
#10247=FACE_OUTER_BOUND('',#16404,.T.);
#10248=FACE_OUTER_BOUND('',#16405,.T.);
#10249=FACE_OUTER_BOUND('',#16406,.T.);
#10250=FACE_OUTER_BOUND('',#16407,.T.);
#10251=FACE_OUTER_BOUND('',#16408,.T.);
#10252=FACE_OUTER_BOUND('',#16409,.T.);
#10253=FACE_OUTER_BOUND('',#16410,.T.);
#10254=FACE_OUTER_BOUND('',#16411,.T.);
#10255=FACE_OUTER_BOUND('',#16412,.T.);
#10256=FACE_OUTER_BOUND('',#16413,.T.);
#10257=FACE_OUTER_BOUND('',#16414,.T.);
#10258=FACE_OUTER_BOUND('',#16415,.T.);
#10259=FACE_OUTER_BOUND('',#16416,.T.);
#10260=FACE_OUTER_BOUND('',#16417,.T.);
#10261=FACE_OUTER_BOUND('',#16418,.T.);
#10262=FACE_OUTER_BOUND('',#16419,.T.);
#10263=FACE_OUTER_BOUND('',#16420,.T.);
#10264=FACE_OUTER_BOUND('',#16421,.T.);
#10265=FACE_OUTER_BOUND('',#16422,.T.);
#10266=FACE_OUTER_BOUND('',#16423,.T.);
#10267=FACE_OUTER_BOUND('',#16424,.T.);
#10268=FACE_OUTER_BOUND('',#16425,.T.);
#10269=FACE_OUTER_BOUND('',#16426,.T.);
#10270=FACE_OUTER_BOUND('',#16427,.T.);
#10271=FACE_OUTER_BOUND('',#16428,.T.);
#10272=FACE_OUTER_BOUND('',#16429,.T.);
#10273=FACE_OUTER_BOUND('',#16430,.T.);
#10274=FACE_OUTER_BOUND('',#16431,.T.);
#10275=FACE_OUTER_BOUND('',#16432,.T.);
#10276=FACE_OUTER_BOUND('',#16433,.T.);
#10277=FACE_OUTER_BOUND('',#16434,.T.);
#10278=FACE_OUTER_BOUND('',#16435,.T.);
#10279=FACE_OUTER_BOUND('',#16436,.T.);
#10280=FACE_OUTER_BOUND('',#16437,.T.);
#10281=FACE_OUTER_BOUND('',#16438,.T.);
#10282=FACE_OUTER_BOUND('',#16439,.T.);
#10283=FACE_OUTER_BOUND('',#16440,.T.);
#10284=FACE_OUTER_BOUND('',#16441,.T.);
#10285=FACE_OUTER_BOUND('',#16442,.T.);
#10286=FACE_OUTER_BOUND('',#16443,.T.);
#10287=FACE_OUTER_BOUND('',#16444,.T.);
#10288=FACE_OUTER_BOUND('',#16445,.T.);
#10289=FACE_OUTER_BOUND('',#16446,.T.);
#10290=FACE_OUTER_BOUND('',#16447,.T.);
#10291=FACE_OUTER_BOUND('',#16448,.T.);
#10292=FACE_OUTER_BOUND('',#16449,.T.);
#10293=FACE_OUTER_BOUND('',#16450,.T.);
#10294=FACE_OUTER_BOUND('',#16451,.T.);
#10295=FACE_OUTER_BOUND('',#16452,.T.);
#10296=FACE_OUTER_BOUND('',#16453,.T.);
#10297=FACE_OUTER_BOUND('',#16454,.T.);
#10298=FACE_OUTER_BOUND('',#16455,.T.);
#10299=FACE_OUTER_BOUND('',#16456,.T.);
#10300=FACE_OUTER_BOUND('',#16457,.T.);
#10301=FACE_OUTER_BOUND('',#16458,.T.);
#10302=FACE_OUTER_BOUND('',#16459,.T.);
#10303=FACE_OUTER_BOUND('',#16460,.T.);
#10304=FACE_OUTER_BOUND('',#16461,.T.);
#10305=FACE_OUTER_BOUND('',#16462,.T.);
#10306=FACE_OUTER_BOUND('',#16463,.T.);
#10307=FACE_OUTER_BOUND('',#16464,.T.);
#10308=FACE_OUTER_BOUND('',#16465,.T.);
#10309=FACE_OUTER_BOUND('',#16466,.T.);
#10310=FACE_OUTER_BOUND('',#16467,.T.);
#10311=FACE_OUTER_BOUND('',#16468,.T.);
#10312=FACE_OUTER_BOUND('',#16469,.T.);
#10313=FACE_OUTER_BOUND('',#16470,.T.);
#10314=FACE_OUTER_BOUND('',#16471,.T.);
#10315=FACE_OUTER_BOUND('',#16472,.T.);
#10316=FACE_OUTER_BOUND('',#16473,.T.);
#10317=FACE_OUTER_BOUND('',#16474,.T.);
#10318=FACE_OUTER_BOUND('',#16475,.T.);
#10319=FACE_OUTER_BOUND('',#16476,.T.);
#10320=FACE_OUTER_BOUND('',#16477,.T.);
#10321=FACE_OUTER_BOUND('',#16478,.T.);
#10322=FACE_OUTER_BOUND('',#16479,.T.);
#10323=FACE_OUTER_BOUND('',#16480,.T.);
#10324=FACE_OUTER_BOUND('',#16481,.T.);
#10325=FACE_OUTER_BOUND('',#16482,.T.);
#10326=FACE_OUTER_BOUND('',#16483,.T.);
#10327=FACE_OUTER_BOUND('',#16484,.T.);
#10328=FACE_OUTER_BOUND('',#16485,.T.);
#10329=FACE_OUTER_BOUND('',#16486,.T.);
#10330=FACE_OUTER_BOUND('',#16487,.T.);
#10331=FACE_OUTER_BOUND('',#16488,.T.);
#10332=FACE_OUTER_BOUND('',#16489,.T.);
#10333=FACE_OUTER_BOUND('',#16490,.T.);
#10334=FACE_OUTER_BOUND('',#16491,.T.);
#10335=FACE_OUTER_BOUND('',#16492,.T.);
#10336=FACE_OUTER_BOUND('',#16493,.T.);
#10337=FACE_OUTER_BOUND('',#16494,.T.);
#10338=FACE_OUTER_BOUND('',#16495,.T.);
#10339=FACE_OUTER_BOUND('',#16496,.T.);
#10340=FACE_OUTER_BOUND('',#16497,.T.);
#10341=FACE_OUTER_BOUND('',#16498,.T.);
#10342=FACE_OUTER_BOUND('',#16499,.T.);
#10343=FACE_OUTER_BOUND('',#16500,.T.);
#10344=FACE_OUTER_BOUND('',#16501,.T.);
#10345=FACE_OUTER_BOUND('',#16502,.T.);
#10346=FACE_OUTER_BOUND('',#16503,.T.);
#10347=FACE_OUTER_BOUND('',#16504,.T.);
#10348=FACE_OUTER_BOUND('',#16505,.T.);
#10349=FACE_OUTER_BOUND('',#16506,.T.);
#10350=FACE_OUTER_BOUND('',#16507,.T.);
#10351=FACE_OUTER_BOUND('',#16508,.T.);
#10352=FACE_OUTER_BOUND('',#16509,.T.);
#10353=FACE_OUTER_BOUND('',#16510,.T.);
#10354=FACE_OUTER_BOUND('',#16511,.T.);
#10355=FACE_OUTER_BOUND('',#16512,.T.);
#10356=FACE_OUTER_BOUND('',#16513,.T.);
#10357=FACE_OUTER_BOUND('',#16514,.T.);
#10358=FACE_OUTER_BOUND('',#16515,.T.);
#10359=FACE_OUTER_BOUND('',#16516,.T.);
#10360=FACE_OUTER_BOUND('',#16517,.T.);
#10361=FACE_OUTER_BOUND('',#16518,.T.);
#10362=FACE_OUTER_BOUND('',#16519,.T.);
#10363=FACE_OUTER_BOUND('',#16520,.T.);
#10364=FACE_OUTER_BOUND('',#16521,.T.);
#10365=FACE_OUTER_BOUND('',#16522,.T.);
#10366=FACE_OUTER_BOUND('',#16523,.T.);
#10367=FACE_OUTER_BOUND('',#16524,.T.);
#10368=FACE_OUTER_BOUND('',#16525,.T.);
#10369=FACE_OUTER_BOUND('',#16526,.T.);
#10370=FACE_OUTER_BOUND('',#16527,.T.);
#10371=FACE_OUTER_BOUND('',#16528,.T.);
#10372=FACE_OUTER_BOUND('',#16529,.T.);
#10373=FACE_OUTER_BOUND('',#16530,.T.);
#10374=FACE_OUTER_BOUND('',#16531,.T.);
#10375=FACE_OUTER_BOUND('',#16532,.T.);
#10376=FACE_OUTER_BOUND('',#16533,.T.);
#10377=FACE_OUTER_BOUND('',#16534,.T.);
#10378=FACE_OUTER_BOUND('',#16535,.T.);
#10379=FACE_OUTER_BOUND('',#16536,.T.);
#10380=FACE_OUTER_BOUND('',#16537,.T.);
#10381=FACE_OUTER_BOUND('',#16538,.T.);
#10382=FACE_OUTER_BOUND('',#16539,.T.);
#10383=FACE_OUTER_BOUND('',#16540,.T.);
#10384=FACE_OUTER_BOUND('',#16541,.T.);
#10385=FACE_OUTER_BOUND('',#16542,.T.);
#10386=FACE_OUTER_BOUND('',#16543,.T.);
#10387=FACE_OUTER_BOUND('',#16544,.T.);
#10388=FACE_OUTER_BOUND('',#16545,.T.);
#10389=FACE_OUTER_BOUND('',#16546,.T.);
#10390=FACE_OUTER_BOUND('',#16547,.T.);
#10391=FACE_OUTER_BOUND('',#16548,.T.);
#10392=FACE_OUTER_BOUND('',#16549,.T.);
#10393=FACE_OUTER_BOUND('',#16550,.T.);
#10394=FACE_OUTER_BOUND('',#16551,.T.);
#10395=FACE_OUTER_BOUND('',#16552,.T.);
#10396=FACE_OUTER_BOUND('',#16553,.T.);
#10397=FACE_OUTER_BOUND('',#16554,.T.);
#10398=FACE_OUTER_BOUND('',#16555,.T.);
#10399=FACE_OUTER_BOUND('',#16556,.T.);
#10400=FACE_OUTER_BOUND('',#16557,.T.);
#10401=FACE_OUTER_BOUND('',#16558,.T.);
#10402=FACE_OUTER_BOUND('',#16559,.T.);
#10403=FACE_OUTER_BOUND('',#16560,.T.);
#10404=FACE_OUTER_BOUND('',#16561,.T.);
#10405=FACE_OUTER_BOUND('',#16562,.T.);
#10406=FACE_OUTER_BOUND('',#16563,.T.);
#10407=FACE_OUTER_BOUND('',#16564,.T.);
#10408=FACE_OUTER_BOUND('',#16565,.T.);
#10409=FACE_OUTER_BOUND('',#16566,.T.);
#10410=FACE_OUTER_BOUND('',#16567,.T.);
#10411=FACE_OUTER_BOUND('',#16568,.T.);
#10412=FACE_OUTER_BOUND('',#16569,.T.);
#10413=FACE_OUTER_BOUND('',#16570,.T.);
#10414=FACE_OUTER_BOUND('',#16571,.T.);
#10415=FACE_OUTER_BOUND('',#16572,.T.);
#10416=FACE_OUTER_BOUND('',#16573,.T.);
#10417=FACE_OUTER_BOUND('',#16574,.T.);
#10418=FACE_OUTER_BOUND('',#16575,.T.);
#10419=FACE_OUTER_BOUND('',#16576,.T.);
#10420=FACE_OUTER_BOUND('',#16577,.T.);
#10421=FACE_OUTER_BOUND('',#16578,.T.);
#10422=FACE_OUTER_BOUND('',#16579,.T.);
#10423=FACE_OUTER_BOUND('',#16580,.T.);
#10424=FACE_OUTER_BOUND('',#16581,.T.);
#10425=FACE_OUTER_BOUND('',#16582,.T.);
#10426=FACE_OUTER_BOUND('',#16583,.T.);
#10427=FACE_OUTER_BOUND('',#16584,.T.);
#10428=FACE_OUTER_BOUND('',#16585,.T.);
#10429=FACE_OUTER_BOUND('',#16586,.T.);
#10430=FACE_OUTER_BOUND('',#16587,.T.);
#10431=FACE_OUTER_BOUND('',#16588,.T.);
#10432=FACE_OUTER_BOUND('',#16589,.T.);
#10433=FACE_OUTER_BOUND('',#16590,.T.);
#10434=FACE_OUTER_BOUND('',#16591,.T.);
#10435=FACE_OUTER_BOUND('',#16592,.T.);
#10436=FACE_OUTER_BOUND('',#16593,.T.);
#10437=FACE_OUTER_BOUND('',#16594,.T.);
#10438=FACE_OUTER_BOUND('',#16595,.T.);
#10439=FACE_OUTER_BOUND('',#16596,.T.);
#10440=FACE_OUTER_BOUND('',#16597,.T.);
#10441=FACE_OUTER_BOUND('',#16598,.T.);
#10442=FACE_OUTER_BOUND('',#16599,.T.);
#10443=FACE_OUTER_BOUND('',#16600,.T.);
#10444=FACE_OUTER_BOUND('',#16601,.T.);
#10445=FACE_OUTER_BOUND('',#16602,.T.);
#10446=FACE_OUTER_BOUND('',#16603,.T.);
#10447=FACE_OUTER_BOUND('',#16604,.T.);
#10448=FACE_OUTER_BOUND('',#16605,.T.);
#10449=FACE_OUTER_BOUND('',#16606,.T.);
#10450=FACE_OUTER_BOUND('',#16607,.T.);
#10451=FACE_OUTER_BOUND('',#16608,.T.);
#10452=FACE_OUTER_BOUND('',#16609,.T.);
#10453=FACE_OUTER_BOUND('',#16610,.T.);
#10454=FACE_OUTER_BOUND('',#16611,.T.);
#10455=FACE_OUTER_BOUND('',#16612,.T.);
#10456=FACE_OUTER_BOUND('',#16613,.T.);
#10457=FACE_OUTER_BOUND('',#16614,.T.);
#10458=FACE_OUTER_BOUND('',#16615,.T.);
#10459=FACE_OUTER_BOUND('',#16616,.T.);
#10460=FACE_OUTER_BOUND('',#16617,.T.);
#10461=FACE_OUTER_BOUND('',#16618,.T.);
#10462=FACE_OUTER_BOUND('',#16619,.T.);
#10463=FACE_OUTER_BOUND('',#16620,.T.);
#10464=FACE_OUTER_BOUND('',#16621,.T.);
#10465=FACE_OUTER_BOUND('',#16622,.T.);
#10466=FACE_OUTER_BOUND('',#16623,.T.);
#10467=FACE_OUTER_BOUND('',#16624,.T.);
#10468=FACE_OUTER_BOUND('',#16625,.T.);
#10469=FACE_OUTER_BOUND('',#16626,.T.);
#10470=FACE_OUTER_BOUND('',#16627,.T.);
#10471=FACE_OUTER_BOUND('',#16628,.T.);
#10472=FACE_OUTER_BOUND('',#16629,.T.);
#10473=FACE_OUTER_BOUND('',#16630,.T.);
#10474=FACE_OUTER_BOUND('',#16631,.T.);
#10475=FACE_OUTER_BOUND('',#16632,.T.);
#10476=FACE_OUTER_BOUND('',#16633,.T.);
#10477=FACE_OUTER_BOUND('',#16634,.T.);
#10478=FACE_OUTER_BOUND('',#16635,.T.);
#10479=FACE_OUTER_BOUND('',#16636,.T.);
#10480=FACE_OUTER_BOUND('',#16637,.T.);
#10481=FACE_OUTER_BOUND('',#16638,.T.);
#10482=FACE_OUTER_BOUND('',#16639,.T.);
#10483=FACE_OUTER_BOUND('',#16640,.T.);
#10484=FACE_OUTER_BOUND('',#16641,.T.);
#10485=FACE_OUTER_BOUND('',#16642,.T.);
#10486=FACE_OUTER_BOUND('',#16643,.T.);
#10487=FACE_OUTER_BOUND('',#16644,.T.);
#10488=FACE_OUTER_BOUND('',#16645,.T.);
#10489=FACE_OUTER_BOUND('',#16646,.T.);
#10490=FACE_OUTER_BOUND('',#16647,.T.);
#10491=FACE_OUTER_BOUND('',#16648,.T.);
#10492=FACE_OUTER_BOUND('',#16649,.T.);
#10493=FACE_OUTER_BOUND('',#16650,.T.);
#10494=FACE_OUTER_BOUND('',#16651,.T.);
#10495=FACE_OUTER_BOUND('',#16652,.T.);
#10496=FACE_OUTER_BOUND('',#16653,.T.);
#10497=FACE_OUTER_BOUND('',#16654,.T.);
#10498=FACE_OUTER_BOUND('',#16655,.T.);
#10499=FACE_OUTER_BOUND('',#16656,.T.);
#10500=FACE_OUTER_BOUND('',#16657,.T.);
#10501=FACE_OUTER_BOUND('',#16658,.T.);
#10502=FACE_OUTER_BOUND('',#16659,.T.);
#10503=FACE_OUTER_BOUND('',#16660,.T.);
#10504=FACE_OUTER_BOUND('',#16661,.T.);
#10505=FACE_OUTER_BOUND('',#16662,.T.);
#10506=FACE_OUTER_BOUND('',#16663,.T.);
#10507=FACE_OUTER_BOUND('',#16664,.T.);
#10508=FACE_OUTER_BOUND('',#16665,.T.);
#10509=FACE_OUTER_BOUND('',#16666,.T.);
#10510=FACE_OUTER_BOUND('',#16667,.T.);
#10511=FACE_OUTER_BOUND('',#16668,.T.);
#10512=FACE_OUTER_BOUND('',#16669,.T.);
#10513=FACE_OUTER_BOUND('',#16670,.T.);
#10514=FACE_OUTER_BOUND('',#16671,.T.);
#10515=FACE_OUTER_BOUND('',#16672,.T.);
#10516=FACE_OUTER_BOUND('',#16673,.T.);
#10517=FACE_OUTER_BOUND('',#16674,.T.);
#10518=FACE_OUTER_BOUND('',#16675,.T.);
#10519=FACE_OUTER_BOUND('',#16676,.T.);
#10520=FACE_OUTER_BOUND('',#16677,.T.);
#10521=FACE_OUTER_BOUND('',#16678,.T.);
#10522=FACE_OUTER_BOUND('',#16679,.T.);
#10523=FACE_OUTER_BOUND('',#16680,.T.);
#10524=FACE_OUTER_BOUND('',#16681,.T.);
#10525=FACE_OUTER_BOUND('',#16682,.T.);
#10526=FACE_OUTER_BOUND('',#16683,.T.);
#10527=FACE_OUTER_BOUND('',#16684,.T.);
#10528=FACE_OUTER_BOUND('',#16685,.T.);
#10529=FACE_OUTER_BOUND('',#16686,.T.);
#10530=FACE_OUTER_BOUND('',#16687,.T.);
#10531=FACE_OUTER_BOUND('',#16688,.T.);
#10532=FACE_OUTER_BOUND('',#16689,.T.);
#10533=FACE_OUTER_BOUND('',#16690,.T.);
#10534=FACE_OUTER_BOUND('',#16691,.T.);
#10535=FACE_OUTER_BOUND('',#16692,.T.);
#10536=FACE_OUTER_BOUND('',#16693,.T.);
#10537=FACE_OUTER_BOUND('',#16694,.T.);
#10538=FACE_OUTER_BOUND('',#16695,.T.);
#10539=FACE_OUTER_BOUND('',#16696,.T.);
#10540=FACE_OUTER_BOUND('',#16697,.T.);
#10541=FACE_OUTER_BOUND('',#16698,.T.);
#10542=FACE_OUTER_BOUND('',#16699,.T.);
#10543=FACE_OUTER_BOUND('',#16700,.T.);
#10544=FACE_OUTER_BOUND('',#16701,.T.);
#10545=FACE_OUTER_BOUND('',#16702,.T.);
#10546=FACE_OUTER_BOUND('',#16703,.T.);
#10547=FACE_OUTER_BOUND('',#16704,.T.);
#10548=FACE_OUTER_BOUND('',#16705,.T.);
#10549=FACE_OUTER_BOUND('',#16706,.T.);
#10550=FACE_OUTER_BOUND('',#16707,.T.);
#10551=FACE_OUTER_BOUND('',#16708,.T.);
#10552=FACE_OUTER_BOUND('',#16709,.T.);
#10553=FACE_OUTER_BOUND('',#16710,.T.);
#10554=FACE_OUTER_BOUND('',#16711,.T.);
#10555=FACE_OUTER_BOUND('',#16712,.T.);
#10556=FACE_OUTER_BOUND('',#16713,.T.);
#10557=FACE_OUTER_BOUND('',#16714,.T.);
#10558=FACE_OUTER_BOUND('',#16715,.T.);
#10559=FACE_OUTER_BOUND('',#16716,.T.);
#10560=FACE_OUTER_BOUND('',#16717,.T.);
#10561=FACE_OUTER_BOUND('',#16718,.T.);
#10562=FACE_OUTER_BOUND('',#16719,.T.);
#10563=FACE_OUTER_BOUND('',#16720,.T.);
#10564=FACE_OUTER_BOUND('',#16721,.T.);
#10565=FACE_OUTER_BOUND('',#16722,.T.);
#10566=FACE_OUTER_BOUND('',#16723,.T.);
#10567=FACE_OUTER_BOUND('',#16724,.T.);
#10568=FACE_OUTER_BOUND('',#16725,.T.);
#10569=FACE_OUTER_BOUND('',#16726,.T.);
#10570=FACE_OUTER_BOUND('',#16727,.T.);
#10571=FACE_OUTER_BOUND('',#16728,.T.);
#10572=FACE_OUTER_BOUND('',#16729,.T.);
#10573=FACE_OUTER_BOUND('',#16730,.T.);
#10574=FACE_OUTER_BOUND('',#16731,.T.);
#10575=FACE_OUTER_BOUND('',#16732,.T.);
#10576=FACE_OUTER_BOUND('',#16733,.T.);
#10577=FACE_OUTER_BOUND('',#16734,.T.);
#10578=FACE_OUTER_BOUND('',#16735,.T.);
#10579=FACE_OUTER_BOUND('',#16736,.T.);
#10580=FACE_OUTER_BOUND('',#16737,.T.);
#10581=FACE_OUTER_BOUND('',#16738,.T.);
#10582=FACE_OUTER_BOUND('',#16739,.T.);
#10583=FACE_OUTER_BOUND('',#16740,.T.);
#10584=FACE_OUTER_BOUND('',#16741,.T.);
#10585=FACE_OUTER_BOUND('',#16742,.T.);
#10586=FACE_OUTER_BOUND('',#16743,.T.);
#10587=FACE_OUTER_BOUND('',#16744,.T.);
#10588=FACE_OUTER_BOUND('',#16745,.T.);
#10589=FACE_OUTER_BOUND('',#16746,.T.);
#10590=FACE_OUTER_BOUND('',#16747,.T.);
#10591=FACE_OUTER_BOUND('',#16748,.T.);
#10592=FACE_OUTER_BOUND('',#16749,.T.);
#10593=FACE_OUTER_BOUND('',#16750,.T.);
#10594=FACE_OUTER_BOUND('',#16751,.T.);
#10595=FACE_OUTER_BOUND('',#16752,.T.);
#10596=FACE_OUTER_BOUND('',#16753,.T.);
#10597=FACE_OUTER_BOUND('',#16754,.T.);
#10598=FACE_OUTER_BOUND('',#16755,.T.);
#10599=FACE_OUTER_BOUND('',#16756,.T.);
#10600=FACE_OUTER_BOUND('',#16757,.T.);
#10601=FACE_OUTER_BOUND('',#16758,.T.);
#10602=FACE_OUTER_BOUND('',#16759,.T.);
#10603=FACE_OUTER_BOUND('',#16760,.T.);
#10604=FACE_OUTER_BOUND('',#16761,.T.);
#10605=FACE_OUTER_BOUND('',#16762,.T.);
#10606=FACE_OUTER_BOUND('',#16763,.T.);
#10607=FACE_OUTER_BOUND('',#16764,.T.);
#10608=FACE_OUTER_BOUND('',#16765,.T.);
#10609=FACE_OUTER_BOUND('',#16766,.T.);
#10610=FACE_OUTER_BOUND('',#16767,.T.);
#10611=FACE_OUTER_BOUND('',#16768,.T.);
#10612=FACE_OUTER_BOUND('',#16769,.T.);
#10613=FACE_OUTER_BOUND('',#16770,.T.);
#10614=FACE_OUTER_BOUND('',#16771,.T.);
#10615=FACE_OUTER_BOUND('',#16772,.T.);
#10616=FACE_OUTER_BOUND('',#16773,.T.);
#10617=FACE_OUTER_BOUND('',#16774,.T.);
#10618=FACE_OUTER_BOUND('',#16775,.T.);
#10619=FACE_OUTER_BOUND('',#16776,.T.);
#10620=FACE_OUTER_BOUND('',#16777,.T.);
#10621=FACE_OUTER_BOUND('',#16778,.T.);
#10622=FACE_OUTER_BOUND('',#16779,.T.);
#10623=FACE_OUTER_BOUND('',#16780,.T.);
#10624=FACE_OUTER_BOUND('',#16781,.T.);
#10625=FACE_OUTER_BOUND('',#16782,.T.);
#10626=FACE_OUTER_BOUND('',#16783,.T.);
#10627=FACE_OUTER_BOUND('',#16784,.T.);
#10628=FACE_OUTER_BOUND('',#16785,.T.);
#10629=FACE_OUTER_BOUND('',#16786,.T.);
#10630=FACE_OUTER_BOUND('',#16787,.T.);
#10631=FACE_OUTER_BOUND('',#16788,.T.);
#10632=FACE_OUTER_BOUND('',#16789,.T.);
#10633=FACE_OUTER_BOUND('',#16790,.T.);
#10634=FACE_OUTER_BOUND('',#16791,.T.);
#10635=FACE_OUTER_BOUND('',#16792,.T.);
#10636=FACE_OUTER_BOUND('',#16793,.T.);
#10637=FACE_OUTER_BOUND('',#16794,.T.);
#10638=FACE_OUTER_BOUND('',#16795,.T.);
#10639=FACE_OUTER_BOUND('',#16796,.T.);
#10640=FACE_OUTER_BOUND('',#16797,.T.);
#10641=FACE_OUTER_BOUND('',#16798,.T.);
#10642=FACE_OUTER_BOUND('',#16799,.T.);
#10643=FACE_OUTER_BOUND('',#16800,.T.);
#10644=FACE_OUTER_BOUND('',#16801,.T.);
#10645=FACE_OUTER_BOUND('',#16802,.T.);
#10646=FACE_OUTER_BOUND('',#16803,.T.);
#10647=FACE_OUTER_BOUND('',#16804,.T.);
#10648=FACE_OUTER_BOUND('',#16805,.T.);
#10649=FACE_OUTER_BOUND('',#16806,.T.);
#10650=FACE_OUTER_BOUND('',#16807,.T.);
#10651=FACE_OUTER_BOUND('',#16808,.T.);
#10652=FACE_OUTER_BOUND('',#16809,.T.);
#10653=FACE_OUTER_BOUND('',#16810,.T.);
#10654=FACE_OUTER_BOUND('',#16811,.T.);
#10655=FACE_OUTER_BOUND('',#16812,.T.);
#10656=FACE_OUTER_BOUND('',#16813,.T.);
#10657=FACE_OUTER_BOUND('',#16814,.T.);
#10658=FACE_OUTER_BOUND('',#16815,.T.);
#10659=FACE_OUTER_BOUND('',#16816,.T.);
#10660=FACE_OUTER_BOUND('',#16817,.T.);
#10661=FACE_OUTER_BOUND('',#16818,.T.);
#10662=FACE_OUTER_BOUND('',#16819,.T.);
#10663=FACE_OUTER_BOUND('',#16820,.T.);
#10664=FACE_OUTER_BOUND('',#16821,.T.);
#10665=FACE_OUTER_BOUND('',#16822,.T.);
#10666=FACE_OUTER_BOUND('',#16823,.T.);
#10667=FACE_OUTER_BOUND('',#16824,.T.);
#10668=FACE_OUTER_BOUND('',#16825,.T.);
#10669=FACE_OUTER_BOUND('',#16826,.T.);
#10670=FACE_OUTER_BOUND('',#16827,.T.);
#10671=FACE_OUTER_BOUND('',#16828,.T.);
#10672=FACE_OUTER_BOUND('',#16829,.T.);
#10673=FACE_OUTER_BOUND('',#16830,.T.);
#10674=FACE_OUTER_BOUND('',#16831,.T.);
#10675=FACE_OUTER_BOUND('',#16832,.T.);
#10676=FACE_OUTER_BOUND('',#16833,.T.);
#10677=FACE_OUTER_BOUND('',#16834,.T.);
#10678=FACE_OUTER_BOUND('',#16835,.T.);
#10679=FACE_OUTER_BOUND('',#16836,.T.);
#10680=FACE_OUTER_BOUND('',#16837,.T.);
#10681=FACE_OUTER_BOUND('',#16838,.T.);
#10682=FACE_OUTER_BOUND('',#16839,.T.);
#10683=FACE_OUTER_BOUND('',#16840,.T.);
#10684=FACE_OUTER_BOUND('',#16841,.T.);
#10685=FACE_OUTER_BOUND('',#16842,.T.);
#10686=FACE_OUTER_BOUND('',#16843,.T.);
#10687=FACE_OUTER_BOUND('',#16844,.T.);
#10688=FACE_OUTER_BOUND('',#16845,.T.);
#10689=FACE_OUTER_BOUND('',#16846,.T.);
#10690=FACE_OUTER_BOUND('',#16847,.T.);
#10691=FACE_OUTER_BOUND('',#16848,.T.);
#10692=FACE_OUTER_BOUND('',#16849,.T.);
#10693=FACE_OUTER_BOUND('',#16850,.T.);
#10694=FACE_OUTER_BOUND('',#16851,.T.);
#10695=FACE_OUTER_BOUND('',#16852,.T.);
#10696=FACE_OUTER_BOUND('',#16853,.T.);
#10697=FACE_OUTER_BOUND('',#16854,.T.);
#10698=FACE_OUTER_BOUND('',#16855,.T.);
#10699=FACE_OUTER_BOUND('',#16856,.T.);
#10700=FACE_OUTER_BOUND('',#16857,.T.);
#10701=FACE_OUTER_BOUND('',#16858,.T.);
#10702=FACE_OUTER_BOUND('',#16859,.T.);
#10703=FACE_OUTER_BOUND('',#16860,.T.);
#10704=FACE_OUTER_BOUND('',#16861,.T.);
#10705=FACE_OUTER_BOUND('',#16862,.T.);
#10706=FACE_OUTER_BOUND('',#16863,.T.);
#10707=FACE_OUTER_BOUND('',#16864,.T.);
#10708=FACE_OUTER_BOUND('',#16865,.T.);
#10709=FACE_OUTER_BOUND('',#16866,.T.);
#10710=FACE_OUTER_BOUND('',#16867,.T.);
#10711=FACE_OUTER_BOUND('',#16868,.T.);
#10712=FACE_OUTER_BOUND('',#16869,.T.);
#10713=FACE_OUTER_BOUND('',#16870,.T.);
#10714=FACE_OUTER_BOUND('',#16871,.T.);
#10715=FACE_OUTER_BOUND('',#16872,.T.);
#10716=FACE_OUTER_BOUND('',#16873,.T.);
#10717=FACE_OUTER_BOUND('',#16874,.T.);
#10718=FACE_OUTER_BOUND('',#16875,.T.);
#10719=FACE_OUTER_BOUND('',#16876,.T.);
#10720=FACE_OUTER_BOUND('',#16877,.T.);
#10721=FACE_OUTER_BOUND('',#16878,.T.);
#10722=FACE_OUTER_BOUND('',#16879,.T.);
#10723=FACE_OUTER_BOUND('',#16880,.T.);
#10724=FACE_OUTER_BOUND('',#16881,.T.);
#10725=FACE_OUTER_BOUND('',#16882,.T.);
#10726=FACE_OUTER_BOUND('',#16883,.T.);
#10727=FACE_OUTER_BOUND('',#16884,.T.);
#10728=FACE_OUTER_BOUND('',#16885,.T.);
#10729=FACE_OUTER_BOUND('',#16886,.T.);
#10730=FACE_OUTER_BOUND('',#16887,.T.);
#10731=FACE_OUTER_BOUND('',#16888,.T.);
#10732=FACE_OUTER_BOUND('',#16889,.T.);
#10733=FACE_OUTER_BOUND('',#16890,.T.);
#10734=FACE_OUTER_BOUND('',#16891,.T.);
#10735=FACE_OUTER_BOUND('',#16892,.T.);
#10736=FACE_OUTER_BOUND('',#16893,.T.);
#10737=FACE_OUTER_BOUND('',#16894,.T.);
#10738=FACE_OUTER_BOUND('',#16895,.T.);
#10739=FACE_OUTER_BOUND('',#16896,.T.);
#10740=FACE_OUTER_BOUND('',#16897,.T.);
#10741=FACE_OUTER_BOUND('',#16898,.T.);
#10742=FACE_OUTER_BOUND('',#16899,.T.);
#10743=FACE_OUTER_BOUND('',#16900,.T.);
#10744=FACE_OUTER_BOUND('',#16901,.T.);
#10745=FACE_OUTER_BOUND('',#16902,.T.);
#10746=FACE_OUTER_BOUND('',#16903,.T.);
#10747=FACE_OUTER_BOUND('',#16904,.T.);
#10748=FACE_OUTER_BOUND('',#16905,.T.);
#10749=FACE_OUTER_BOUND('',#16906,.T.);
#10750=FACE_OUTER_BOUND('',#16907,.T.);
#10751=FACE_OUTER_BOUND('',#16908,.T.);
#10752=FACE_OUTER_BOUND('',#16909,.T.);
#10753=FACE_OUTER_BOUND('',#16910,.T.);
#10754=FACE_OUTER_BOUND('',#16911,.T.);
#10755=FACE_OUTER_BOUND('',#16912,.T.);
#10756=FACE_OUTER_BOUND('',#16913,.T.);
#10757=FACE_OUTER_BOUND('',#16914,.T.);
#10758=FACE_OUTER_BOUND('',#16915,.T.);
#10759=FACE_OUTER_BOUND('',#16916,.T.);
#10760=FACE_OUTER_BOUND('',#16917,.T.);
#10761=FACE_OUTER_BOUND('',#16918,.T.);
#10762=FACE_OUTER_BOUND('',#16919,.T.);
#10763=FACE_OUTER_BOUND('',#16920,.T.);
#10764=FACE_OUTER_BOUND('',#16921,.T.);
#10765=FACE_OUTER_BOUND('',#16922,.T.);
#10766=FACE_OUTER_BOUND('',#16923,.T.);
#10767=FACE_OUTER_BOUND('',#16924,.T.);
#10768=FACE_OUTER_BOUND('',#16925,.T.);
#10769=FACE_OUTER_BOUND('',#16926,.T.);
#10770=FACE_OUTER_BOUND('',#16927,.T.);
#10771=FACE_OUTER_BOUND('',#16928,.T.);
#10772=FACE_OUTER_BOUND('',#16929,.T.);
#10773=FACE_OUTER_BOUND('',#16930,.T.);
#10774=FACE_OUTER_BOUND('',#16931,.T.);
#10775=FACE_OUTER_BOUND('',#16932,.T.);
#10776=FACE_OUTER_BOUND('',#16933,.T.);
#10777=FACE_OUTER_BOUND('',#16934,.T.);
#10778=FACE_OUTER_BOUND('',#16935,.T.);
#10779=FACE_OUTER_BOUND('',#16936,.T.);
#10780=FACE_OUTER_BOUND('',#16937,.T.);
#10781=FACE_OUTER_BOUND('',#16938,.T.);
#10782=FACE_OUTER_BOUND('',#16939,.T.);
#10783=FACE_OUTER_BOUND('',#16940,.T.);
#10784=FACE_OUTER_BOUND('',#16941,.T.);
#10785=FACE_OUTER_BOUND('',#16942,.T.);
#10786=FACE_OUTER_BOUND('',#16943,.T.);
#10787=FACE_OUTER_BOUND('',#16944,.T.);
#10788=FACE_OUTER_BOUND('',#16945,.T.);
#10789=FACE_OUTER_BOUND('',#16946,.T.);
#10790=FACE_OUTER_BOUND('',#16947,.T.);
#10791=FACE_OUTER_BOUND('',#16948,.T.);
#10792=FACE_OUTER_BOUND('',#16949,.T.);
#10793=FACE_OUTER_BOUND('',#16950,.T.);
#10794=FACE_OUTER_BOUND('',#16951,.T.);
#10795=FACE_OUTER_BOUND('',#16952,.T.);
#10796=FACE_OUTER_BOUND('',#16953,.T.);
#10797=FACE_OUTER_BOUND('',#16954,.T.);
#10798=FACE_OUTER_BOUND('',#16955,.T.);
#10799=FACE_OUTER_BOUND('',#16956,.T.);
#10800=FACE_OUTER_BOUND('',#16957,.T.);
#10801=FACE_OUTER_BOUND('',#16958,.T.);
#10802=FACE_OUTER_BOUND('',#16959,.T.);
#10803=FACE_OUTER_BOUND('',#16960,.T.);
#10804=FACE_OUTER_BOUND('',#16961,.T.);
#10805=FACE_OUTER_BOUND('',#16962,.T.);
#10806=FACE_OUTER_BOUND('',#16963,.T.);
#10807=FACE_OUTER_BOUND('',#16964,.T.);
#10808=FACE_OUTER_BOUND('',#16965,.T.);
#10809=FACE_OUTER_BOUND('',#16966,.T.);
#10810=FACE_OUTER_BOUND('',#16967,.T.);
#10811=FACE_OUTER_BOUND('',#16968,.T.);
#10812=FACE_OUTER_BOUND('',#16969,.T.);
#10813=FACE_OUTER_BOUND('',#16970,.T.);
#10814=FACE_OUTER_BOUND('',#16971,.T.);
#10815=FACE_OUTER_BOUND('',#16972,.T.);
#10816=FACE_OUTER_BOUND('',#16973,.T.);
#10817=FACE_OUTER_BOUND('',#16974,.T.);
#10818=FACE_OUTER_BOUND('',#16975,.T.);
#10819=FACE_OUTER_BOUND('',#16976,.T.);
#10820=FACE_OUTER_BOUND('',#16977,.T.);
#10821=FACE_OUTER_BOUND('',#16978,.T.);
#10822=FACE_OUTER_BOUND('',#16979,.T.);
#10823=FACE_OUTER_BOUND('',#16980,.T.);
#10824=FACE_OUTER_BOUND('',#16981,.T.);
#10825=FACE_OUTER_BOUND('',#16982,.T.);
#10826=FACE_OUTER_BOUND('',#16983,.T.);
#10827=FACE_OUTER_BOUND('',#16984,.T.);
#10828=FACE_OUTER_BOUND('',#16985,.T.);
#10829=FACE_OUTER_BOUND('',#16986,.T.);
#10830=FACE_OUTER_BOUND('',#16987,.T.);
#10831=FACE_OUTER_BOUND('',#16988,.T.);
#10832=FACE_OUTER_BOUND('',#16989,.T.);
#10833=FACE_OUTER_BOUND('',#16990,.T.);
#10834=FACE_OUTER_BOUND('',#16991,.T.);
#10835=FACE_OUTER_BOUND('',#16992,.T.);
#10836=FACE_OUTER_BOUND('',#16993,.T.);
#10837=FACE_OUTER_BOUND('',#16994,.T.);
#10838=FACE_OUTER_BOUND('',#16995,.T.);
#10839=FACE_OUTER_BOUND('',#16996,.T.);
#10840=FACE_OUTER_BOUND('',#16997,.T.);
#10841=FACE_OUTER_BOUND('',#16998,.T.);
#10842=FACE_OUTER_BOUND('',#16999,.T.);
#10843=FACE_OUTER_BOUND('',#17000,.T.);
#10844=FACE_OUTER_BOUND('',#17001,.T.);
#10845=FACE_OUTER_BOUND('',#17002,.T.);
#10846=FACE_OUTER_BOUND('',#17003,.T.);
#10847=FACE_OUTER_BOUND('',#17004,.T.);
#10848=FACE_OUTER_BOUND('',#17005,.T.);
#10849=FACE_OUTER_BOUND('',#17006,.T.);
#10850=FACE_OUTER_BOUND('',#17007,.T.);
#10851=FACE_OUTER_BOUND('',#17008,.T.);
#10852=FACE_OUTER_BOUND('',#17009,.T.);
#10853=FACE_OUTER_BOUND('',#17010,.T.);
#10854=FACE_OUTER_BOUND('',#17012,.T.);
#10855=FACE_OUTER_BOUND('',#17013,.T.);
#10856=FACE_OUTER_BOUND('',#17014,.T.);
#10857=FACE_OUTER_BOUND('',#17015,.T.);
#10858=FACE_OUTER_BOUND('',#17016,.T.);
#10859=FACE_OUTER_BOUND('',#17017,.T.);
#10860=FACE_OUTER_BOUND('',#17019,.T.);
#10861=FACE_OUTER_BOUND('',#17021,.T.);
#10862=FACE_OUTER_BOUND('',#17022,.T.);
#10863=FACE_OUTER_BOUND('',#17023,.T.);
#10864=FACE_OUTER_BOUND('',#17024,.T.);
#10865=FACE_OUTER_BOUND('',#17025,.T.);
#10866=FACE_OUTER_BOUND('',#17026,.T.);
#10867=FACE_OUTER_BOUND('',#17027,.T.);
#10868=FACE_OUTER_BOUND('',#17028,.T.);
#10869=FACE_OUTER_BOUND('',#17029,.T.);
#10870=FACE_OUTER_BOUND('',#17030,.T.);
#10871=FACE_OUTER_BOUND('',#17031,.T.);
#10872=FACE_OUTER_BOUND('',#17032,.T.);
#10873=FACE_OUTER_BOUND('',#17033,.T.);
#10874=FACE_OUTER_BOUND('',#17034,.T.);
#10875=FACE_OUTER_BOUND('',#17035,.T.);
#10876=FACE_OUTER_BOUND('',#17036,.T.);
#10877=FACE_OUTER_BOUND('',#17037,.T.);
#10878=FACE_OUTER_BOUND('',#17038,.T.);
#10879=FACE_OUTER_BOUND('',#17039,.T.);
#10880=FACE_OUTER_BOUND('',#17040,.T.);
#10881=FACE_OUTER_BOUND('',#17041,.T.);
#10882=FACE_OUTER_BOUND('',#17042,.T.);
#10883=FACE_OUTER_BOUND('',#17043,.T.);
#10884=FACE_OUTER_BOUND('',#17044,.T.);
#10885=FACE_OUTER_BOUND('',#17045,.T.);
#10886=FACE_OUTER_BOUND('',#17046,.T.);
#10887=FACE_OUTER_BOUND('',#17047,.T.);
#10888=FACE_OUTER_BOUND('',#17048,.T.);
#10889=FACE_OUTER_BOUND('',#17049,.T.);
#10890=FACE_OUTER_BOUND('',#17050,.T.);
#10891=FACE_OUTER_BOUND('',#17051,.T.);
#10892=FACE_OUTER_BOUND('',#17052,.T.);
#10893=FACE_OUTER_BOUND('',#17053,.T.);
#10894=FACE_OUTER_BOUND('',#17054,.T.);
#10895=FACE_OUTER_BOUND('',#17055,.T.);
#10896=FACE_OUTER_BOUND('',#17056,.T.);
#10897=FACE_OUTER_BOUND('',#17057,.T.);
#10898=FACE_OUTER_BOUND('',#17058,.T.);
#10899=FACE_OUTER_BOUND('',#17059,.T.);
#10900=FACE_OUTER_BOUND('',#17060,.T.);
#10901=FACE_OUTER_BOUND('',#17061,.T.);
#10902=FACE_OUTER_BOUND('',#17062,.T.);
#10903=FACE_OUTER_BOUND('',#17063,.T.);
#10904=FACE_OUTER_BOUND('',#17064,.T.);
#10905=FACE_OUTER_BOUND('',#17065,.T.);
#10906=FACE_OUTER_BOUND('',#17066,.T.);
#10907=FACE_OUTER_BOUND('',#17067,.T.);
#10908=FACE_OUTER_BOUND('',#17068,.T.);
#10909=FACE_OUTER_BOUND('',#17069,.T.);
#10910=FACE_OUTER_BOUND('',#17070,.T.);
#10911=FACE_OUTER_BOUND('',#17071,.T.);
#10912=FACE_OUTER_BOUND('',#17072,.T.);
#10913=FACE_OUTER_BOUND('',#17073,.T.);
#10914=FACE_OUTER_BOUND('',#17074,.T.);
#10915=FACE_OUTER_BOUND('',#17075,.T.);
#10916=FACE_OUTER_BOUND('',#17076,.T.);
#10917=FACE_OUTER_BOUND('',#17077,.T.);
#10918=FACE_OUTER_BOUND('',#17078,.T.);
#10919=FACE_OUTER_BOUND('',#17079,.T.);
#10920=FACE_OUTER_BOUND('',#17080,.T.);
#10921=FACE_OUTER_BOUND('',#17081,.T.);
#10922=FACE_OUTER_BOUND('',#17082,.T.);
#10923=FACE_OUTER_BOUND('',#17083,.T.);
#10924=FACE_OUTER_BOUND('',#17084,.T.);
#10925=FACE_OUTER_BOUND('',#17085,.T.);
#10926=FACE_OUTER_BOUND('',#17086,.T.);
#10927=FACE_OUTER_BOUND('',#17087,.T.);
#10928=FACE_OUTER_BOUND('',#17088,.T.);
#10929=FACE_OUTER_BOUND('',#17089,.T.);
#10930=FACE_OUTER_BOUND('',#17090,.T.);
#10931=FACE_OUTER_BOUND('',#17091,.T.);
#10932=FACE_OUTER_BOUND('',#17092,.T.);
#10933=FACE_OUTER_BOUND('',#17093,.T.);
#10934=FACE_OUTER_BOUND('',#17094,.T.);
#10935=FACE_OUTER_BOUND('',#17095,.T.);
#10936=FACE_OUTER_BOUND('',#17096,.T.);
#10937=FACE_OUTER_BOUND('',#17097,.T.);
#10938=FACE_OUTER_BOUND('',#17098,.T.);
#10939=FACE_OUTER_BOUND('',#17099,.T.);
#10940=FACE_OUTER_BOUND('',#17100,.T.);
#10941=FACE_OUTER_BOUND('',#17101,.T.);
#10942=FACE_OUTER_BOUND('',#17102,.T.);
#10943=FACE_OUTER_BOUND('',#17103,.T.);
#10944=FACE_OUTER_BOUND('',#17104,.T.);
#10945=FACE_OUTER_BOUND('',#17105,.T.);
#10946=FACE_OUTER_BOUND('',#17106,.T.);
#10947=FACE_OUTER_BOUND('',#17107,.T.);
#10948=FACE_OUTER_BOUND('',#17108,.T.);
#10949=FACE_OUTER_BOUND('',#17109,.T.);
#10950=FACE_OUTER_BOUND('',#17110,.T.);
#10951=FACE_OUTER_BOUND('',#17111,.T.);
#10952=FACE_OUTER_BOUND('',#17112,.T.);
#10953=FACE_OUTER_BOUND('',#17113,.T.);
#10954=FACE_OUTER_BOUND('',#17114,.T.);
#10955=FACE_OUTER_BOUND('',#17115,.T.);
#10956=FACE_OUTER_BOUND('',#17116,.T.);
#10957=FACE_OUTER_BOUND('',#17117,.T.);
#10958=FACE_OUTER_BOUND('',#17118,.T.);
#10959=FACE_OUTER_BOUND('',#17119,.T.);
#10960=FACE_OUTER_BOUND('',#17120,.T.);
#10961=FACE_OUTER_BOUND('',#17121,.T.);
#10962=FACE_OUTER_BOUND('',#17122,.T.);
#10963=FACE_OUTER_BOUND('',#17123,.T.);
#10964=FACE_OUTER_BOUND('',#17124,.T.);
#10965=FACE_OUTER_BOUND('',#17125,.T.);
#10966=FACE_OUTER_BOUND('',#17126,.T.);
#10967=FACE_OUTER_BOUND('',#17127,.T.);
#10968=FACE_OUTER_BOUND('',#17128,.T.);
#10969=FACE_OUTER_BOUND('',#17129,.T.);
#10970=FACE_OUTER_BOUND('',#17130,.T.);
#10971=FACE_OUTER_BOUND('',#17131,.T.);
#10972=FACE_OUTER_BOUND('',#17132,.T.);
#10973=FACE_OUTER_BOUND('',#17133,.T.);
#10974=FACE_OUTER_BOUND('',#17134,.T.);
#10975=FACE_OUTER_BOUND('',#17135,.T.);
#10976=FACE_OUTER_BOUND('',#17136,.T.);
#10977=FACE_OUTER_BOUND('',#17137,.T.);
#10978=FACE_OUTER_BOUND('',#17138,.T.);
#10979=FACE_OUTER_BOUND('',#17139,.T.);
#10980=FACE_OUTER_BOUND('',#17140,.T.);
#10981=FACE_OUTER_BOUND('',#17141,.T.);
#10982=FACE_OUTER_BOUND('',#17142,.T.);
#10983=FACE_OUTER_BOUND('',#17143,.T.);
#10984=FACE_OUTER_BOUND('',#17144,.T.);
#10985=FACE_OUTER_BOUND('',#17145,.T.);
#10986=FACE_OUTER_BOUND('',#17146,.T.);
#10987=FACE_OUTER_BOUND('',#17147,.T.);
#10988=FACE_OUTER_BOUND('',#17148,.T.);
#10989=FACE_OUTER_BOUND('',#17149,.T.);
#10990=FACE_OUTER_BOUND('',#17150,.T.);
#10991=FACE_OUTER_BOUND('',#17151,.T.);
#10992=FACE_OUTER_BOUND('',#17152,.T.);
#10993=FACE_OUTER_BOUND('',#17153,.T.);
#10994=FACE_OUTER_BOUND('',#17154,.T.);
#10995=FACE_OUTER_BOUND('',#17155,.T.);
#10996=FACE_OUTER_BOUND('',#17156,.T.);
#10997=FACE_OUTER_BOUND('',#17157,.T.);
#10998=FACE_OUTER_BOUND('',#17158,.T.);
#10999=FACE_OUTER_BOUND('',#17159,.T.);
#11000=FACE_OUTER_BOUND('',#17160,.T.);
#11001=FACE_OUTER_BOUND('',#17161,.T.);
#11002=FACE_OUTER_BOUND('',#17162,.T.);
#11003=FACE_OUTER_BOUND('',#17163,.T.);
#11004=FACE_OUTER_BOUND('',#17164,.T.);
#11005=FACE_OUTER_BOUND('',#17165,.T.);
#11006=FACE_OUTER_BOUND('',#17166,.T.);
#11007=FACE_OUTER_BOUND('',#17167,.T.);
#11008=FACE_OUTER_BOUND('',#17168,.T.);
#11009=FACE_OUTER_BOUND('',#17169,.T.);
#11010=FACE_OUTER_BOUND('',#17170,.T.);
#11011=FACE_OUTER_BOUND('',#17171,.T.);
#11012=FACE_OUTER_BOUND('',#17172,.T.);
#11013=FACE_OUTER_BOUND('',#17173,.T.);
#11014=FACE_OUTER_BOUND('',#17174,.T.);
#11015=FACE_OUTER_BOUND('',#17175,.T.);
#11016=FACE_OUTER_BOUND('',#17176,.T.);
#11017=FACE_OUTER_BOUND('',#17177,.T.);
#11018=FACE_OUTER_BOUND('',#17178,.T.);
#11019=FACE_OUTER_BOUND('',#17179,.T.);
#11020=FACE_OUTER_BOUND('',#17180,.T.);
#11021=FACE_OUTER_BOUND('',#17181,.T.);
#11022=FACE_OUTER_BOUND('',#17182,.T.);
#11023=FACE_OUTER_BOUND('',#17183,.T.);
#11024=FACE_OUTER_BOUND('',#17184,.T.);
#11025=FACE_OUTER_BOUND('',#17185,.T.);
#11026=FACE_OUTER_BOUND('',#17186,.T.);
#11027=FACE_OUTER_BOUND('',#17187,.T.);
#11028=FACE_OUTER_BOUND('',#17188,.T.);
#11029=FACE_OUTER_BOUND('',#17189,.T.);
#11030=FACE_OUTER_BOUND('',#17190,.T.);
#11031=FACE_OUTER_BOUND('',#17191,.T.);
#11032=FACE_OUTER_BOUND('',#17192,.T.);
#11033=FACE_OUTER_BOUND('',#17193,.T.);
#11034=FACE_OUTER_BOUND('',#17194,.T.);
#11035=FACE_OUTER_BOUND('',#17195,.T.);
#11036=FACE_OUTER_BOUND('',#17196,.T.);
#11037=FACE_OUTER_BOUND('',#17197,.T.);
#11038=FACE_OUTER_BOUND('',#17198,.T.);
#11039=FACE_OUTER_BOUND('',#17199,.T.);
#11040=FACE_OUTER_BOUND('',#17200,.T.);
#11041=FACE_OUTER_BOUND('',#17201,.T.);
#11042=FACE_OUTER_BOUND('',#17202,.T.);
#11043=FACE_OUTER_BOUND('',#17203,.T.);
#11044=FACE_OUTER_BOUND('',#17204,.T.);
#11045=FACE_OUTER_BOUND('',#17205,.T.);
#11046=FACE_OUTER_BOUND('',#17206,.T.);
#11047=FACE_OUTER_BOUND('',#17207,.T.);
#11048=FACE_OUTER_BOUND('',#17208,.T.);
#11049=FACE_OUTER_BOUND('',#17209,.T.);
#11050=FACE_OUTER_BOUND('',#17210,.T.);
#11051=FACE_OUTER_BOUND('',#17211,.T.);
#11052=FACE_OUTER_BOUND('',#17212,.T.);
#11053=FACE_OUTER_BOUND('',#17213,.T.);
#11054=FACE_OUTER_BOUND('',#17214,.T.);
#11055=FACE_OUTER_BOUND('',#17215,.T.);
#11056=FACE_OUTER_BOUND('',#17216,.T.);
#11057=FACE_OUTER_BOUND('',#17217,.T.);
#11058=FACE_OUTER_BOUND('',#17218,.T.);
#11059=FACE_OUTER_BOUND('',#17219,.T.);
#11060=FACE_OUTER_BOUND('',#17220,.T.);
#11061=FACE_OUTER_BOUND('',#17221,.T.);
#11062=FACE_OUTER_BOUND('',#17222,.T.);
#11063=FACE_OUTER_BOUND('',#17223,.T.);
#11064=FACE_OUTER_BOUND('',#17224,.T.);
#11065=FACE_OUTER_BOUND('',#17225,.T.);
#11066=FACE_OUTER_BOUND('',#17226,.T.);
#11067=FACE_OUTER_BOUND('',#17227,.T.);
#11068=FACE_OUTER_BOUND('',#17228,.T.);
#11069=FACE_OUTER_BOUND('',#17229,.T.);
#11070=FACE_OUTER_BOUND('',#17230,.T.);
#11071=FACE_OUTER_BOUND('',#17231,.T.);
#11072=FACE_OUTER_BOUND('',#17232,.T.);
#11073=FACE_OUTER_BOUND('',#17233,.T.);
#11074=FACE_OUTER_BOUND('',#17234,.T.);
#11075=FACE_OUTER_BOUND('',#17235,.T.);
#11076=FACE_OUTER_BOUND('',#17236,.T.);
#11077=FACE_OUTER_BOUND('',#17237,.T.);
#11078=FACE_OUTER_BOUND('',#17238,.T.);
#11079=FACE_OUTER_BOUND('',#17239,.T.);
#11080=FACE_OUTER_BOUND('',#17240,.T.);
#11081=FACE_OUTER_BOUND('',#17241,.T.);
#11082=FACE_OUTER_BOUND('',#17242,.T.);
#11083=FACE_OUTER_BOUND('',#17243,.T.);
#11084=FACE_OUTER_BOUND('',#17244,.T.);
#11085=FACE_OUTER_BOUND('',#17245,.T.);
#11086=FACE_OUTER_BOUND('',#17246,.T.);
#11087=FACE_OUTER_BOUND('',#17247,.T.);
#11088=FACE_OUTER_BOUND('',#17248,.T.);
#11089=FACE_OUTER_BOUND('',#17249,.T.);
#11090=FACE_OUTER_BOUND('',#17250,.T.);
#11091=FACE_OUTER_BOUND('',#17251,.T.);
#11092=FACE_OUTER_BOUND('',#17252,.T.);
#11093=FACE_OUTER_BOUND('',#17253,.T.);
#11094=FACE_OUTER_BOUND('',#17254,.T.);
#11095=FACE_OUTER_BOUND('',#17255,.T.);
#11096=FACE_OUTER_BOUND('',#17256,.T.);
#11097=FACE_OUTER_BOUND('',#17257,.T.);
#11098=FACE_OUTER_BOUND('',#17258,.T.);
#11099=FACE_OUTER_BOUND('',#17259,.T.);
#11100=FACE_OUTER_BOUND('',#17260,.T.);
#11101=FACE_OUTER_BOUND('',#17261,.T.);
#11102=FACE_OUTER_BOUND('',#17262,.T.);
#11103=FACE_OUTER_BOUND('',#17263,.T.);
#11104=FACE_OUTER_BOUND('',#17264,.T.);
#11105=FACE_OUTER_BOUND('',#17265,.T.);
#11106=FACE_OUTER_BOUND('',#17266,.T.);
#11107=FACE_OUTER_BOUND('',#17267,.T.);
#11108=FACE_OUTER_BOUND('',#17268,.T.);
#11109=FACE_OUTER_BOUND('',#17269,.T.);
#11110=FACE_OUTER_BOUND('',#17270,.T.);
#11111=FACE_OUTER_BOUND('',#17271,.T.);
#11112=FACE_OUTER_BOUND('',#17272,.T.);
#11113=FACE_OUTER_BOUND('',#17273,.T.);
#11114=FACE_OUTER_BOUND('',#17274,.T.);
#11115=FACE_OUTER_BOUND('',#17275,.T.);
#11116=FACE_OUTER_BOUND('',#17276,.T.);
#11117=FACE_OUTER_BOUND('',#17277,.T.);
#11118=FACE_OUTER_BOUND('',#17278,.T.);
#11119=FACE_OUTER_BOUND('',#17279,.T.);
#11120=FACE_OUTER_BOUND('',#17280,.T.);
#11121=FACE_OUTER_BOUND('',#17281,.T.);
#11122=FACE_OUTER_BOUND('',#17282,.T.);
#11123=FACE_OUTER_BOUND('',#17283,.T.);
#11124=FACE_OUTER_BOUND('',#17284,.T.);
#11125=FACE_OUTER_BOUND('',#17285,.T.);
#11126=FACE_OUTER_BOUND('',#17286,.T.);
#11127=FACE_OUTER_BOUND('',#17287,.T.);
#11128=FACE_OUTER_BOUND('',#17288,.T.);
#11129=FACE_OUTER_BOUND('',#17289,.T.);
#11130=FACE_OUTER_BOUND('',#17290,.T.);
#11131=FACE_OUTER_BOUND('',#17291,.T.);
#11132=FACE_OUTER_BOUND('',#17292,.T.);
#11133=FACE_OUTER_BOUND('',#17293,.T.);
#11134=FACE_OUTER_BOUND('',#17294,.T.);
#11135=FACE_OUTER_BOUND('',#17295,.T.);
#11136=FACE_OUTER_BOUND('',#17296,.T.);
#11137=FACE_OUTER_BOUND('',#17297,.T.);
#11138=FACE_OUTER_BOUND('',#17298,.T.);
#11139=FACE_OUTER_BOUND('',#17299,.T.);
#11140=FACE_OUTER_BOUND('',#17300,.T.);
#11141=FACE_OUTER_BOUND('',#17301,.T.);
#11142=FACE_OUTER_BOUND('',#17302,.T.);
#11143=FACE_OUTER_BOUND('',#17303,.T.);
#11144=FACE_OUTER_BOUND('',#17304,.T.);
#11145=FACE_OUTER_BOUND('',#17305,.T.);
#11146=FACE_OUTER_BOUND('',#17306,.T.);
#11147=FACE_OUTER_BOUND('',#17307,.T.);
#11148=FACE_OUTER_BOUND('',#17308,.T.);
#11149=FACE_OUTER_BOUND('',#17309,.T.);
#11150=FACE_OUTER_BOUND('',#17310,.T.);
#11151=FACE_OUTER_BOUND('',#17311,.T.);
#11152=FACE_OUTER_BOUND('',#17312,.T.);
#11153=FACE_OUTER_BOUND('',#17313,.T.);
#11154=FACE_OUTER_BOUND('',#17314,.T.);
#11155=FACE_OUTER_BOUND('',#17315,.T.);
#11156=FACE_OUTER_BOUND('',#17316,.T.);
#11157=FACE_OUTER_BOUND('',#17317,.T.);
#11158=FACE_OUTER_BOUND('',#17318,.T.);
#11159=FACE_OUTER_BOUND('',#17319,.T.);
#11160=FACE_OUTER_BOUND('',#17320,.T.);
#11161=FACE_OUTER_BOUND('',#17321,.T.);
#11162=FACE_OUTER_BOUND('',#17322,.T.);
#11163=FACE_OUTER_BOUND('',#17323,.T.);
#11164=FACE_OUTER_BOUND('',#17324,.T.);
#11165=FACE_OUTER_BOUND('',#17325,.T.);
#11166=FACE_OUTER_BOUND('',#17326,.T.);
#11167=FACE_OUTER_BOUND('',#17327,.T.);
#11168=FACE_OUTER_BOUND('',#17328,.T.);
#11169=FACE_OUTER_BOUND('',#17329,.T.);
#11170=FACE_OUTER_BOUND('',#17330,.T.);
#11171=FACE_OUTER_BOUND('',#17331,.T.);
#11172=FACE_OUTER_BOUND('',#17332,.T.);
#11173=FACE_OUTER_BOUND('',#17333,.T.);
#11174=FACE_OUTER_BOUND('',#17334,.T.);
#11175=FACE_OUTER_BOUND('',#17335,.T.);
#11176=FACE_OUTER_BOUND('',#17336,.T.);
#11177=FACE_OUTER_BOUND('',#17337,.T.);
#11178=FACE_OUTER_BOUND('',#17338,.T.);
#11179=FACE_OUTER_BOUND('',#17339,.T.);
#11180=FACE_OUTER_BOUND('',#17340,.T.);
#11181=FACE_OUTER_BOUND('',#17341,.T.);
#11182=FACE_OUTER_BOUND('',#17342,.T.);
#11183=FACE_OUTER_BOUND('',#17343,.T.);
#11184=FACE_OUTER_BOUND('',#17344,.T.);
#11185=FACE_OUTER_BOUND('',#17345,.T.);
#11186=FACE_OUTER_BOUND('',#17346,.T.);
#11187=FACE_OUTER_BOUND('',#17347,.T.);
#11188=FACE_OUTER_BOUND('',#17348,.T.);
#11189=FACE_OUTER_BOUND('',#17349,.T.);
#11190=FACE_OUTER_BOUND('',#17350,.T.);
#11191=FACE_OUTER_BOUND('',#17351,.T.);
#11192=FACE_OUTER_BOUND('',#17352,.T.);
#11193=FACE_OUTER_BOUND('',#17353,.T.);
#11194=FACE_OUTER_BOUND('',#17354,.T.);
#11195=FACE_OUTER_BOUND('',#17355,.T.);
#11196=FACE_OUTER_BOUND('',#17356,.T.);
#11197=FACE_OUTER_BOUND('',#17357,.T.);
#11198=FACE_OUTER_BOUND('',#17358,.T.);
#11199=FACE_OUTER_BOUND('',#17359,.T.);
#11200=FACE_OUTER_BOUND('',#17360,.T.);
#11201=FACE_OUTER_BOUND('',#17361,.T.);
#11202=FACE_OUTER_BOUND('',#17362,.T.);
#11203=FACE_OUTER_BOUND('',#17363,.T.);
#11204=FACE_OUTER_BOUND('',#17364,.T.);
#11205=FACE_OUTER_BOUND('',#17365,.T.);
#11206=FACE_OUTER_BOUND('',#17366,.T.);
#11207=FACE_OUTER_BOUND('',#17367,.T.);
#11208=FACE_OUTER_BOUND('',#17368,.T.);
#11209=FACE_OUTER_BOUND('',#17369,.T.);
#11210=FACE_OUTER_BOUND('',#17370,.T.);
#11211=FACE_OUTER_BOUND('',#17371,.T.);
#11212=FACE_OUTER_BOUND('',#17372,.T.);
#11213=FACE_OUTER_BOUND('',#17373,.T.);
#11214=FACE_OUTER_BOUND('',#17374,.T.);
#11215=FACE_OUTER_BOUND('',#17375,.T.);
#11216=FACE_OUTER_BOUND('',#17376,.T.);
#11217=FACE_OUTER_BOUND('',#17377,.T.);
#11218=FACE_OUTER_BOUND('',#17378,.T.);
#11219=FACE_OUTER_BOUND('',#17379,.T.);
#11220=FACE_OUTER_BOUND('',#17380,.T.);
#11221=FACE_OUTER_BOUND('',#17381,.T.);
#11222=FACE_OUTER_BOUND('',#17382,.T.);
#11223=FACE_OUTER_BOUND('',#17383,.T.);
#11224=FACE_OUTER_BOUND('',#17384,.T.);
#11225=FACE_OUTER_BOUND('',#17385,.T.);
#11226=FACE_OUTER_BOUND('',#17386,.T.);
#11227=FACE_OUTER_BOUND('',#17387,.T.);
#11228=FACE_OUTER_BOUND('',#17388,.T.);
#11229=FACE_OUTER_BOUND('',#17389,.T.);
#11230=FACE_OUTER_BOUND('',#17390,.T.);
#11231=FACE_OUTER_BOUND('',#17391,.T.);
#11232=FACE_OUTER_BOUND('',#17392,.T.);
#11233=FACE_OUTER_BOUND('',#17393,.T.);
#11234=FACE_OUTER_BOUND('',#17394,.T.);
#11235=FACE_OUTER_BOUND('',#17395,.T.);
#11236=FACE_OUTER_BOUND('',#17396,.T.);
#11237=FACE_OUTER_BOUND('',#17397,.T.);
#11238=FACE_OUTER_BOUND('',#17398,.T.);
#11239=FACE_OUTER_BOUND('',#17399,.T.);
#11240=FACE_OUTER_BOUND('',#17400,.T.);
#11241=FACE_OUTER_BOUND('',#17401,.T.);
#11242=FACE_OUTER_BOUND('',#17402,.T.);
#11243=FACE_OUTER_BOUND('',#17403,.T.);
#11244=FACE_OUTER_BOUND('',#17404,.T.);
#11245=FACE_OUTER_BOUND('',#17405,.T.);
#11246=FACE_OUTER_BOUND('',#17406,.T.);
#11247=FACE_OUTER_BOUND('',#17407,.T.);
#11248=FACE_OUTER_BOUND('',#17408,.T.);
#11249=FACE_OUTER_BOUND('',#17409,.T.);
#11250=FACE_OUTER_BOUND('',#17410,.T.);
#11251=FACE_OUTER_BOUND('',#17411,.T.);
#11252=FACE_OUTER_BOUND('',#17412,.T.);
#11253=FACE_OUTER_BOUND('',#17413,.T.);
#11254=FACE_OUTER_BOUND('',#17414,.T.);
#11255=FACE_OUTER_BOUND('',#17415,.T.);
#11256=FACE_OUTER_BOUND('',#17416,.T.);
#11257=FACE_OUTER_BOUND('',#17417,.T.);
#11258=FACE_OUTER_BOUND('',#17418,.T.);
#11259=FACE_OUTER_BOUND('',#17419,.T.);
#11260=FACE_OUTER_BOUND('',#17420,.T.);
#11261=FACE_OUTER_BOUND('',#17421,.T.);
#11262=FACE_OUTER_BOUND('',#17422,.T.);
#11263=FACE_OUTER_BOUND('',#17423,.T.);
#11264=FACE_OUTER_BOUND('',#17424,.T.);
#11265=FACE_OUTER_BOUND('',#17425,.T.);
#11266=FACE_OUTER_BOUND('',#17426,.T.);
#11267=FACE_OUTER_BOUND('',#17427,.T.);
#11268=FACE_OUTER_BOUND('',#17428,.T.);
#11269=FACE_OUTER_BOUND('',#17429,.T.);
#11270=FACE_OUTER_BOUND('',#17430,.T.);
#11271=FACE_OUTER_BOUND('',#17431,.T.);
#11272=FACE_OUTER_BOUND('',#17432,.T.);
#11273=FACE_OUTER_BOUND('',#17433,.T.);
#11274=FACE_OUTER_BOUND('',#17434,.T.);
#11275=FACE_OUTER_BOUND('',#17435,.T.);
#11276=FACE_OUTER_BOUND('',#17436,.T.);
#11277=FACE_OUTER_BOUND('',#17437,.T.);
#11278=FACE_OUTER_BOUND('',#17438,.T.);
#11279=FACE_OUTER_BOUND('',#17439,.T.);
#11280=FACE_OUTER_BOUND('',#17440,.T.);
#11281=FACE_OUTER_BOUND('',#17441,.T.);
#11282=FACE_OUTER_BOUND('',#17442,.T.);
#11283=FACE_OUTER_BOUND('',#17443,.T.);
#11284=FACE_OUTER_BOUND('',#17444,.T.);
#11285=FACE_OUTER_BOUND('',#17445,.T.);
#11286=FACE_OUTER_BOUND('',#17446,.T.);
#11287=FACE_OUTER_BOUND('',#17447,.T.);
#11288=FACE_OUTER_BOUND('',#17448,.T.);
#11289=FACE_OUTER_BOUND('',#17449,.T.);
#11290=FACE_OUTER_BOUND('',#17450,.T.);
#11291=FACE_OUTER_BOUND('',#17451,.T.);
#11292=FACE_OUTER_BOUND('',#17452,.T.);
#11293=FACE_OUTER_BOUND('',#17453,.T.);
#11294=FACE_OUTER_BOUND('',#17454,.T.);
#11295=FACE_OUTER_BOUND('',#17455,.T.);
#11296=FACE_OUTER_BOUND('',#17456,.T.);
#11297=FACE_OUTER_BOUND('',#17457,.T.);
#11298=FACE_OUTER_BOUND('',#17458,.T.);
#11299=FACE_OUTER_BOUND('',#17459,.T.);
#11300=FACE_OUTER_BOUND('',#17460,.T.);
#11301=FACE_OUTER_BOUND('',#17461,.T.);
#11302=FACE_OUTER_BOUND('',#17462,.T.);
#11303=FACE_OUTER_BOUND('',#17463,.T.);
#11304=FACE_OUTER_BOUND('',#17464,.T.);
#11305=FACE_OUTER_BOUND('',#17465,.T.);
#11306=FACE_OUTER_BOUND('',#17466,.T.);
#11307=FACE_OUTER_BOUND('',#17467,.T.);
#11308=FACE_OUTER_BOUND('',#17468,.T.);
#11309=FACE_OUTER_BOUND('',#17469,.T.);
#11310=FACE_OUTER_BOUND('',#17470,.T.);
#11311=FACE_OUTER_BOUND('',#17471,.T.);
#11312=FACE_OUTER_BOUND('',#17472,.T.);
#11313=FACE_OUTER_BOUND('',#17473,.T.);
#11314=FACE_OUTER_BOUND('',#17474,.T.);
#11315=FACE_OUTER_BOUND('',#17475,.T.);
#11316=FACE_OUTER_BOUND('',#17476,.T.);
#11317=FACE_OUTER_BOUND('',#17477,.T.);
#11318=FACE_OUTER_BOUND('',#17478,.T.);
#11319=FACE_OUTER_BOUND('',#17479,.T.);
#11320=FACE_OUTER_BOUND('',#17480,.T.);
#11321=FACE_OUTER_BOUND('',#17481,.T.);
#11322=FACE_OUTER_BOUND('',#17482,.T.);
#11323=FACE_OUTER_BOUND('',#17483,.T.);
#11324=FACE_OUTER_BOUND('',#17484,.T.);
#11325=FACE_OUTER_BOUND('',#17485,.T.);
#11326=FACE_OUTER_BOUND('',#17486,.T.);
#11327=FACE_OUTER_BOUND('',#17487,.T.);
#11328=FACE_OUTER_BOUND('',#17488,.T.);
#11329=FACE_OUTER_BOUND('',#17489,.T.);
#11330=FACE_OUTER_BOUND('',#17490,.T.);
#11331=FACE_OUTER_BOUND('',#17491,.T.);
#11332=FACE_OUTER_BOUND('',#17492,.T.);
#11333=FACE_OUTER_BOUND('',#17493,.T.);
#11334=FACE_OUTER_BOUND('',#17494,.T.);
#11335=FACE_OUTER_BOUND('',#17495,.T.);
#11336=FACE_OUTER_BOUND('',#17496,.T.);
#11337=FACE_OUTER_BOUND('',#17497,.T.);
#11338=FACE_OUTER_BOUND('',#17498,.T.);
#11339=FACE_OUTER_BOUND('',#17499,.T.);
#11340=FACE_OUTER_BOUND('',#17500,.T.);
#11341=FACE_OUTER_BOUND('',#17501,.T.);
#11342=FACE_OUTER_BOUND('',#17502,.T.);
#11343=FACE_OUTER_BOUND('',#17503,.T.);
#11344=FACE_OUTER_BOUND('',#17504,.T.);
#11345=FACE_OUTER_BOUND('',#17505,.T.);
#11346=FACE_OUTER_BOUND('',#17506,.T.);
#11347=FACE_OUTER_BOUND('',#17507,.T.);
#11348=FACE_OUTER_BOUND('',#17508,.T.);
#11349=FACE_OUTER_BOUND('',#17509,.T.);
#11350=FACE_OUTER_BOUND('',#17510,.T.);
#11351=FACE_OUTER_BOUND('',#17511,.T.);
#11352=FACE_OUTER_BOUND('',#17512,.T.);
#11353=FACE_OUTER_BOUND('',#17513,.T.);
#11354=FACE_OUTER_BOUND('',#17514,.T.);
#11355=FACE_OUTER_BOUND('',#17515,.T.);
#11356=FACE_OUTER_BOUND('',#17516,.T.);
#11357=FACE_OUTER_BOUND('',#17517,.T.);
#11358=FACE_OUTER_BOUND('',#17518,.T.);
#11359=FACE_OUTER_BOUND('',#17519,.T.);
#11360=FACE_OUTER_BOUND('',#17520,.T.);
#11361=FACE_OUTER_BOUND('',#17521,.T.);
#11362=FACE_OUTER_BOUND('',#17522,.T.);
#11363=FACE_OUTER_BOUND('',#17523,.T.);
#11364=FACE_OUTER_BOUND('',#17524,.T.);
#11365=FACE_OUTER_BOUND('',#17525,.T.);
#11366=FACE_OUTER_BOUND('',#17526,.T.);
#11367=FACE_OUTER_BOUND('',#17527,.T.);
#11368=FACE_OUTER_BOUND('',#17528,.T.);
#11369=FACE_OUTER_BOUND('',#17529,.T.);
#11370=FACE_OUTER_BOUND('',#17530,.T.);
#11371=FACE_OUTER_BOUND('',#17531,.T.);
#11372=FACE_OUTER_BOUND('',#17532,.T.);
#11373=FACE_OUTER_BOUND('',#17533,.T.);
#11374=FACE_OUTER_BOUND('',#17534,.T.);
#11375=FACE_OUTER_BOUND('',#17535,.T.);
#11376=FACE_OUTER_BOUND('',#17536,.T.);
#11377=FACE_OUTER_BOUND('',#17537,.T.);
#11378=FACE_OUTER_BOUND('',#17538,.T.);
#11379=FACE_OUTER_BOUND('',#17539,.T.);
#11380=FACE_OUTER_BOUND('',#17540,.T.);
#11381=FACE_OUTER_BOUND('',#17541,.T.);
#11382=FACE_OUTER_BOUND('',#17542,.T.);
#11383=FACE_OUTER_BOUND('',#17543,.T.);
#11384=FACE_OUTER_BOUND('',#17544,.T.);
#11385=FACE_OUTER_BOUND('',#17545,.T.);
#11386=FACE_OUTER_BOUND('',#17546,.T.);
#11387=FACE_OUTER_BOUND('',#17547,.T.);
#11388=FACE_OUTER_BOUND('',#17548,.T.);
#11389=FACE_OUTER_BOUND('',#17549,.T.);
#11390=FACE_OUTER_BOUND('',#17550,.T.);
#11391=FACE_OUTER_BOUND('',#17551,.T.);
#11392=FACE_OUTER_BOUND('',#17552,.T.);
#11393=FACE_OUTER_BOUND('',#17553,.T.);
#11394=FACE_OUTER_BOUND('',#17554,.T.);
#11395=FACE_OUTER_BOUND('',#17555,.T.);
#11396=FACE_OUTER_BOUND('',#17556,.T.);
#11397=FACE_OUTER_BOUND('',#17557,.T.);
#11398=FACE_OUTER_BOUND('',#17558,.T.);
#11399=FACE_OUTER_BOUND('',#17559,.T.);
#11400=FACE_OUTER_BOUND('',#17560,.T.);
#11401=FACE_OUTER_BOUND('',#17561,.T.);
#11402=FACE_OUTER_BOUND('',#17562,.T.);
#11403=FACE_OUTER_BOUND('',#17563,.T.);
#11404=FACE_OUTER_BOUND('',#17564,.T.);
#11405=FACE_OUTER_BOUND('',#17565,.T.);
#11406=FACE_OUTER_BOUND('',#17566,.T.);
#11407=FACE_OUTER_BOUND('',#17567,.T.);
#11408=FACE_OUTER_BOUND('',#17568,.T.);
#11409=FACE_OUTER_BOUND('',#17569,.T.);
#11410=FACE_OUTER_BOUND('',#17570,.T.);
#11411=FACE_OUTER_BOUND('',#17571,.T.);
#11412=FACE_OUTER_BOUND('',#17572,.T.);
#11413=FACE_OUTER_BOUND('',#17573,.T.);
#11414=FACE_OUTER_BOUND('',#17574,.T.);
#11415=FACE_OUTER_BOUND('',#17575,.T.);
#11416=FACE_OUTER_BOUND('',#17576,.T.);
#11417=FACE_OUTER_BOUND('',#17577,.T.);
#11418=FACE_OUTER_BOUND('',#17578,.T.);
#11419=FACE_OUTER_BOUND('',#17579,.T.);
#11420=FACE_OUTER_BOUND('',#17580,.T.);
#11421=FACE_OUTER_BOUND('',#17581,.T.);
#11422=FACE_OUTER_BOUND('',#17582,.T.);
#11423=FACE_OUTER_BOUND('',#17583,.T.);
#11424=FACE_OUTER_BOUND('',#17584,.T.);
#11425=FACE_OUTER_BOUND('',#17585,.T.);
#11426=FACE_OUTER_BOUND('',#17586,.T.);
#11427=FACE_OUTER_BOUND('',#17587,.T.);
#11428=FACE_OUTER_BOUND('',#17588,.T.);
#11429=FACE_OUTER_BOUND('',#17589,.T.);
#11430=FACE_OUTER_BOUND('',#17590,.T.);
#11431=FACE_OUTER_BOUND('',#17591,.T.);
#11432=FACE_OUTER_BOUND('',#17592,.T.);
#11433=FACE_OUTER_BOUND('',#17593,.T.);
#11434=FACE_OUTER_BOUND('',#17594,.T.);
#11435=FACE_OUTER_BOUND('',#17595,.T.);
#11436=FACE_OUTER_BOUND('',#17596,.T.);
#11437=FACE_OUTER_BOUND('',#17597,.T.);
#11438=FACE_OUTER_BOUND('',#17598,.T.);
#11439=FACE_OUTER_BOUND('',#17599,.T.);
#11440=FACE_OUTER_BOUND('',#17600,.T.);
#11441=FACE_OUTER_BOUND('',#17601,.T.);
#11442=FACE_OUTER_BOUND('',#17602,.T.);
#11443=FACE_OUTER_BOUND('',#17603,.T.);
#11444=FACE_OUTER_BOUND('',#17604,.T.);
#11445=FACE_OUTER_BOUND('',#17605,.T.);
#11446=FACE_OUTER_BOUND('',#17606,.T.);
#11447=FACE_OUTER_BOUND('',#17607,.T.);
#11448=FACE_OUTER_BOUND('',#17608,.T.);
#11449=FACE_OUTER_BOUND('',#17609,.T.);
#11450=FACE_OUTER_BOUND('',#17610,.T.);
#11451=FACE_OUTER_BOUND('',#17611,.T.);
#11452=FACE_OUTER_BOUND('',#17612,.T.);
#11453=FACE_OUTER_BOUND('',#17613,.T.);
#11454=FACE_OUTER_BOUND('',#17614,.T.);
#11455=FACE_OUTER_BOUND('',#17615,.T.);
#11456=FACE_OUTER_BOUND('',#17616,.T.);
#11457=FACE_OUTER_BOUND('',#17617,.T.);
#11458=FACE_OUTER_BOUND('',#17618,.T.);
#11459=FACE_OUTER_BOUND('',#17619,.T.);
#11460=FACE_OUTER_BOUND('',#17620,.T.);
#11461=FACE_OUTER_BOUND('',#17621,.T.);
#11462=FACE_OUTER_BOUND('',#17622,.T.);
#11463=FACE_OUTER_BOUND('',#17623,.T.);
#11464=FACE_OUTER_BOUND('',#17624,.T.);
#11465=FACE_OUTER_BOUND('',#17625,.T.);
#11466=FACE_OUTER_BOUND('',#17626,.T.);
#11467=FACE_OUTER_BOUND('',#17627,.T.);
#11468=FACE_OUTER_BOUND('',#17628,.T.);
#11469=FACE_OUTER_BOUND('',#17629,.T.);
#11470=FACE_OUTER_BOUND('',#17630,.T.);
#11471=FACE_OUTER_BOUND('',#17631,.T.);
#11472=FACE_OUTER_BOUND('',#17632,.T.);
#11473=FACE_OUTER_BOUND('',#17633,.T.);
#11474=FACE_OUTER_BOUND('',#17634,.T.);
#11475=FACE_OUTER_BOUND('',#17635,.T.);
#11476=FACE_OUTER_BOUND('',#17636,.T.);
#11477=FACE_OUTER_BOUND('',#17637,.T.);
#11478=FACE_OUTER_BOUND('',#17638,.T.);
#11479=FACE_OUTER_BOUND('',#17639,.T.);
#11480=FACE_OUTER_BOUND('',#17640,.T.);
#11481=FACE_OUTER_BOUND('',#17641,.T.);
#11482=FACE_OUTER_BOUND('',#17642,.T.);
#11483=FACE_OUTER_BOUND('',#17643,.T.);
#11484=FACE_OUTER_BOUND('',#17644,.T.);
#11485=FACE_OUTER_BOUND('',#17645,.T.);
#11486=FACE_OUTER_BOUND('',#17646,.T.);
#11487=FACE_OUTER_BOUND('',#17647,.T.);
#11488=FACE_OUTER_BOUND('',#17648,.T.);
#11489=FACE_OUTER_BOUND('',#17649,.T.);
#11490=FACE_OUTER_BOUND('',#17650,.T.);
#11491=FACE_OUTER_BOUND('',#17651,.T.);
#11492=FACE_OUTER_BOUND('',#17652,.T.);
#11493=FACE_OUTER_BOUND('',#17653,.T.);
#11494=FACE_OUTER_BOUND('',#17654,.T.);
#11495=FACE_OUTER_BOUND('',#17655,.T.);
#11496=FACE_OUTER_BOUND('',#17656,.T.);
#11497=FACE_OUTER_BOUND('',#17657,.T.);
#11498=FACE_OUTER_BOUND('',#17658,.T.);
#11499=FACE_OUTER_BOUND('',#17659,.T.);
#11500=FACE_OUTER_BOUND('',#17660,.T.);
#11501=FACE_OUTER_BOUND('',#17661,.T.);
#11502=FACE_OUTER_BOUND('',#17662,.T.);
#11503=FACE_OUTER_BOUND('',#17663,.T.);
#11504=FACE_OUTER_BOUND('',#17664,.T.);
#11505=FACE_OUTER_BOUND('',#17665,.T.);
#11506=FACE_OUTER_BOUND('',#17666,.T.);
#11507=FACE_OUTER_BOUND('',#17667,.T.);
#11508=FACE_OUTER_BOUND('',#17668,.T.);
#11509=FACE_OUTER_BOUND('',#17669,.T.);
#11510=FACE_OUTER_BOUND('',#17670,.T.);
#11511=FACE_OUTER_BOUND('',#17671,.T.);
#11512=FACE_OUTER_BOUND('',#17672,.T.);
#11513=FACE_OUTER_BOUND('',#17673,.T.);
#11514=FACE_OUTER_BOUND('',#17674,.T.);
#11515=FACE_OUTER_BOUND('',#17675,.T.);
#11516=FACE_OUTER_BOUND('',#17676,.T.);
#11517=FACE_OUTER_BOUND('',#17677,.T.);
#11518=FACE_OUTER_BOUND('',#17678,.T.);
#11519=FACE_OUTER_BOUND('',#17679,.T.);
#11520=FACE_OUTER_BOUND('',#17680,.T.);
#11521=FACE_OUTER_BOUND('',#17681,.T.);
#11522=FACE_OUTER_BOUND('',#17682,.T.);
#11523=FACE_OUTER_BOUND('',#17683,.T.);
#11524=FACE_OUTER_BOUND('',#17684,.T.);
#11525=FACE_OUTER_BOUND('',#17685,.T.);
#11526=FACE_OUTER_BOUND('',#17686,.T.);
#11527=FACE_OUTER_BOUND('',#17687,.T.);
#11528=FACE_OUTER_BOUND('',#17688,.T.);
#11529=FACE_OUTER_BOUND('',#17689,.T.);
#11530=FACE_OUTER_BOUND('',#17690,.T.);
#11531=FACE_OUTER_BOUND('',#17691,.T.);
#11532=FACE_OUTER_BOUND('',#17692,.T.);
#11533=FACE_OUTER_BOUND('',#17693,.T.);
#11534=FACE_OUTER_BOUND('',#17694,.T.);
#11535=FACE_OUTER_BOUND('',#17695,.T.);
#11536=FACE_OUTER_BOUND('',#17696,.T.);
#11537=FACE_OUTER_BOUND('',#17697,.T.);
#11538=FACE_OUTER_BOUND('',#17698,.T.);
#11539=FACE_OUTER_BOUND('',#17699,.T.);
#11540=FACE_OUTER_BOUND('',#17700,.T.);
#11541=FACE_OUTER_BOUND('',#17701,.T.);
#11542=FACE_OUTER_BOUND('',#17702,.T.);
#11543=FACE_OUTER_BOUND('',#17703,.T.);
#11544=FACE_OUTER_BOUND('',#17704,.T.);
#11545=FACE_OUTER_BOUND('',#17705,.T.);
#11546=FACE_OUTER_BOUND('',#17706,.T.);
#11547=FACE_OUTER_BOUND('',#17707,.T.);
#11548=FACE_OUTER_BOUND('',#17708,.T.);
#11549=FACE_OUTER_BOUND('',#17709,.T.);
#11550=FACE_OUTER_BOUND('',#17710,.T.);
#11551=FACE_OUTER_BOUND('',#17711,.T.);
#11552=FACE_OUTER_BOUND('',#17712,.T.);
#11553=FACE_OUTER_BOUND('',#17713,.T.);
#11554=FACE_OUTER_BOUND('',#17714,.T.);
#11555=FACE_OUTER_BOUND('',#17715,.T.);
#11556=FACE_OUTER_BOUND('',#17716,.T.);
#11557=FACE_OUTER_BOUND('',#17717,.T.);
#11558=FACE_OUTER_BOUND('',#17718,.T.);
#11559=FACE_OUTER_BOUND('',#17719,.T.);
#11560=FACE_OUTER_BOUND('',#17720,.T.);
#11561=FACE_OUTER_BOUND('',#17721,.T.);
#11562=FACE_OUTER_BOUND('',#17722,.T.);
#11563=FACE_OUTER_BOUND('',#17723,.T.);
#11564=FACE_OUTER_BOUND('',#17724,.T.);
#11565=FACE_OUTER_BOUND('',#17725,.T.);
#11566=FACE_OUTER_BOUND('',#17726,.T.);
#11567=FACE_OUTER_BOUND('',#17727,.T.);
#11568=FACE_OUTER_BOUND('',#17728,.T.);
#11569=FACE_OUTER_BOUND('',#17729,.T.);
#11570=FACE_OUTER_BOUND('',#17730,.T.);
#11571=FACE_OUTER_BOUND('',#17731,.T.);
#11572=FACE_OUTER_BOUND('',#17732,.T.);
#11573=FACE_OUTER_BOUND('',#17733,.T.);
#11574=FACE_OUTER_BOUND('',#17734,.T.);
#11575=FACE_OUTER_BOUND('',#17735,.T.);
#11576=FACE_OUTER_BOUND('',#17736,.T.);
#11577=FACE_OUTER_BOUND('',#17737,.T.);
#11578=FACE_OUTER_BOUND('',#17738,.T.);
#11579=FACE_OUTER_BOUND('',#17739,.T.);
#11580=FACE_OUTER_BOUND('',#17740,.T.);
#11581=FACE_OUTER_BOUND('',#17741,.T.);
#11582=FACE_OUTER_BOUND('',#17742,.T.);
#11583=FACE_OUTER_BOUND('',#17743,.T.);
#11584=FACE_OUTER_BOUND('',#17744,.T.);
#11585=FACE_OUTER_BOUND('',#17745,.T.);
#11586=FACE_OUTER_BOUND('',#17746,.T.);
#11587=FACE_OUTER_BOUND('',#17747,.T.);
#11588=FACE_OUTER_BOUND('',#17748,.T.);
#11589=FACE_OUTER_BOUND('',#17749,.T.);
#11590=FACE_OUTER_BOUND('',#17750,.T.);
#11591=FACE_OUTER_BOUND('',#17751,.T.);
#11592=FACE_OUTER_BOUND('',#17752,.T.);
#11593=FACE_OUTER_BOUND('',#17753,.T.);
#11594=FACE_OUTER_BOUND('',#17754,.T.);
#11595=FACE_OUTER_BOUND('',#17755,.T.);
#11596=FACE_OUTER_BOUND('',#17756,.T.);
#11597=FACE_OUTER_BOUND('',#17757,.T.);
#11598=FACE_OUTER_BOUND('',#17758,.T.);
#11599=FACE_OUTER_BOUND('',#17759,.T.);
#11600=FACE_OUTER_BOUND('',#17760,.T.);
#11601=FACE_OUTER_BOUND('',#17761,.T.);
#11602=FACE_OUTER_BOUND('',#17762,.T.);
#11603=FACE_OUTER_BOUND('',#17763,.T.);
#11604=FACE_OUTER_BOUND('',#17764,.T.);
#11605=FACE_OUTER_BOUND('',#17765,.T.);
#11606=FACE_OUTER_BOUND('',#17766,.T.);
#11607=FACE_OUTER_BOUND('',#17767,.T.);
#11608=FACE_OUTER_BOUND('',#17768,.T.);
#11609=FACE_OUTER_BOUND('',#17769,.T.);
#11610=FACE_OUTER_BOUND('',#17770,.T.);
#11611=FACE_OUTER_BOUND('',#17771,.T.);
#11612=FACE_OUTER_BOUND('',#17772,.T.);
#11613=FACE_OUTER_BOUND('',#17773,.T.);
#11614=FACE_OUTER_BOUND('',#17774,.T.);
#11615=FACE_OUTER_BOUND('',#17775,.T.);
#11616=FACE_OUTER_BOUND('',#17776,.T.);
#11617=FACE_OUTER_BOUND('',#17777,.T.);
#11618=FACE_OUTER_BOUND('',#17778,.T.);
#11619=FACE_OUTER_BOUND('',#17779,.T.);
#11620=FACE_OUTER_BOUND('',#17780,.T.);
#11621=FACE_OUTER_BOUND('',#17781,.T.);
#11622=FACE_OUTER_BOUND('',#17782,.T.);
#11623=FACE_OUTER_BOUND('',#17783,.T.);
#11624=FACE_OUTER_BOUND('',#17784,.T.);
#11625=FACE_OUTER_BOUND('',#17785,.T.);
#11626=FACE_OUTER_BOUND('',#17786,.T.);
#11627=FACE_OUTER_BOUND('',#17787,.T.);
#11628=FACE_OUTER_BOUND('',#17788,.T.);
#11629=FACE_OUTER_BOUND('',#17789,.T.);
#11630=FACE_OUTER_BOUND('',#17790,.T.);
#11631=FACE_OUTER_BOUND('',#17791,.T.);
#11632=FACE_OUTER_BOUND('',#17792,.T.);
#11633=FACE_OUTER_BOUND('',#17793,.T.);
#11634=FACE_OUTER_BOUND('',#17794,.T.);
#11635=FACE_OUTER_BOUND('',#17795,.T.);
#11636=FACE_OUTER_BOUND('',#17796,.T.);
#11637=FACE_OUTER_BOUND('',#17797,.T.);
#11638=FACE_OUTER_BOUND('',#17798,.T.);
#11639=FACE_OUTER_BOUND('',#17799,.T.);
#11640=FACE_OUTER_BOUND('',#17800,.T.);
#11641=FACE_OUTER_BOUND('',#17801,.T.);
#11642=FACE_OUTER_BOUND('',#17802,.T.);
#11643=FACE_OUTER_BOUND('',#17803,.T.);
#11644=FACE_OUTER_BOUND('',#17804,.T.);
#11645=FACE_OUTER_BOUND('',#17805,.T.);
#11646=FACE_OUTER_BOUND('',#17806,.T.);
#11647=FACE_OUTER_BOUND('',#17807,.T.);
#11648=FACE_OUTER_BOUND('',#17808,.T.);
#11649=FACE_OUTER_BOUND('',#17809,.T.);
#11650=FACE_OUTER_BOUND('',#17810,.T.);
#11651=FACE_OUTER_BOUND('',#17811,.T.);
#11652=FACE_OUTER_BOUND('',#17812,.T.);
#11653=FACE_OUTER_BOUND('',#17813,.T.);
#11654=FACE_OUTER_BOUND('',#17814,.T.);
#11655=FACE_OUTER_BOUND('',#17815,.T.);
#11656=FACE_OUTER_BOUND('',#17816,.T.);
#11657=FACE_OUTER_BOUND('',#17817,.T.);
#11658=FACE_OUTER_BOUND('',#17818,.T.);
#11659=FACE_OUTER_BOUND('',#17819,.T.);
#11660=FACE_OUTER_BOUND('',#17820,.T.);
#11661=FACE_OUTER_BOUND('',#17821,.T.);
#11662=FACE_OUTER_BOUND('',#17822,.T.);
#11663=FACE_OUTER_BOUND('',#17823,.T.);
#11664=FACE_OUTER_BOUND('',#17824,.T.);
#11665=FACE_OUTER_BOUND('',#17825,.T.);
#11666=FACE_OUTER_BOUND('',#17826,.T.);
#11667=FACE_OUTER_BOUND('',#17827,.T.);
#11668=FACE_OUTER_BOUND('',#17828,.T.);
#11669=FACE_OUTER_BOUND('',#17829,.T.);
#11670=FACE_OUTER_BOUND('',#17830,.T.);
#11671=FACE_OUTER_BOUND('',#17831,.T.);
#11672=FACE_OUTER_BOUND('',#17832,.T.);
#11673=FACE_OUTER_BOUND('',#17833,.T.);
#11674=FACE_OUTER_BOUND('',#17834,.T.);
#11675=FACE_OUTER_BOUND('',#17835,.T.);
#11676=FACE_OUTER_BOUND('',#17836,.T.);
#11677=FACE_OUTER_BOUND('',#17837,.T.);
#11678=FACE_OUTER_BOUND('',#17838,.T.);
#11679=FACE_OUTER_BOUND('',#17839,.T.);
#11680=FACE_OUTER_BOUND('',#17840,.T.);
#11681=FACE_OUTER_BOUND('',#17841,.T.);
#11682=FACE_OUTER_BOUND('',#17842,.T.);
#11683=FACE_OUTER_BOUND('',#17843,.T.);
#11684=FACE_OUTER_BOUND('',#17844,.T.);
#11685=FACE_OUTER_BOUND('',#17845,.T.);
#11686=FACE_OUTER_BOUND('',#17846,.T.);
#11687=FACE_OUTER_BOUND('',#17847,.T.);
#11688=FACE_OUTER_BOUND('',#17848,.T.);
#11689=FACE_OUTER_BOUND('',#17849,.T.);
#11690=FACE_OUTER_BOUND('',#17850,.T.);
#11691=FACE_OUTER_BOUND('',#17851,.T.);
#11692=FACE_OUTER_BOUND('',#17852,.T.);
#11693=FACE_OUTER_BOUND('',#17853,.T.);
#11694=FACE_OUTER_BOUND('',#17854,.T.);
#11695=FACE_OUTER_BOUND('',#17855,.T.);
#11696=FACE_OUTER_BOUND('',#17856,.T.);
#11697=FACE_OUTER_BOUND('',#17857,.T.);
#11698=FACE_OUTER_BOUND('',#17858,.T.);
#11699=FACE_OUTER_BOUND('',#17859,.T.);
#11700=FACE_OUTER_BOUND('',#17860,.T.);
#11701=FACE_OUTER_BOUND('',#17861,.T.);
#11702=FACE_OUTER_BOUND('',#17862,.T.);
#11703=FACE_OUTER_BOUND('',#17863,.T.);
#11704=FACE_OUTER_BOUND('',#17864,.T.);
#11705=FACE_OUTER_BOUND('',#17865,.T.);
#11706=FACE_OUTER_BOUND('',#17866,.T.);
#11707=FACE_OUTER_BOUND('',#17867,.T.);
#11708=FACE_OUTER_BOUND('',#17868,.T.);
#11709=FACE_OUTER_BOUND('',#17869,.T.);
#11710=FACE_OUTER_BOUND('',#17870,.T.);
#11711=FACE_OUTER_BOUND('',#17871,.T.);
#11712=FACE_OUTER_BOUND('',#17872,.T.);
#11713=FACE_OUTER_BOUND('',#17873,.T.);
#11714=FACE_OUTER_BOUND('',#17874,.T.);
#11715=FACE_OUTER_BOUND('',#17875,.T.);
#11716=FACE_OUTER_BOUND('',#17876,.T.);
#11717=FACE_OUTER_BOUND('',#17877,.T.);
#11718=FACE_OUTER_BOUND('',#17878,.T.);
#11719=FACE_OUTER_BOUND('',#17879,.T.);
#11720=FACE_OUTER_BOUND('',#17880,.T.);
#11721=FACE_OUTER_BOUND('',#17881,.T.);
#11722=FACE_OUTER_BOUND('',#17882,.T.);
#11723=FACE_OUTER_BOUND('',#17883,.T.);
#11724=FACE_OUTER_BOUND('',#17884,.T.);
#11725=FACE_OUTER_BOUND('',#17885,.T.);
#11726=FACE_OUTER_BOUND('',#17886,.T.);
#11727=FACE_OUTER_BOUND('',#17887,.T.);
#11728=FACE_OUTER_BOUND('',#17888,.T.);
#11729=FACE_OUTER_BOUND('',#17889,.T.);
#11730=FACE_OUTER_BOUND('',#17890,.T.);
#11731=FACE_OUTER_BOUND('',#17891,.T.);
#11732=FACE_OUTER_BOUND('',#17892,.T.);
#11733=FACE_OUTER_BOUND('',#17893,.T.);
#11734=FACE_OUTER_BOUND('',#17894,.T.);
#11735=FACE_OUTER_BOUND('',#17895,.T.);
#11736=FACE_OUTER_BOUND('',#17896,.T.);
#11737=FACE_OUTER_BOUND('',#17897,.T.);
#11738=FACE_OUTER_BOUND('',#17898,.T.);
#11739=FACE_OUTER_BOUND('',#17899,.T.);
#11740=FACE_OUTER_BOUND('',#17900,.T.);
#11741=FACE_OUTER_BOUND('',#17901,.T.);
#11742=FACE_OUTER_BOUND('',#17902,.T.);
#11743=FACE_OUTER_BOUND('',#17903,.T.);
#11744=FACE_OUTER_BOUND('',#17904,.T.);
#11745=FACE_OUTER_BOUND('',#17905,.T.);
#11746=FACE_OUTER_BOUND('',#17906,.T.);
#11747=FACE_OUTER_BOUND('',#17907,.T.);
#11748=FACE_OUTER_BOUND('',#17908,.T.);
#11749=FACE_OUTER_BOUND('',#17909,.T.);
#11750=FACE_OUTER_BOUND('',#17910,.T.);
#11751=FACE_OUTER_BOUND('',#17911,.T.);
#11752=FACE_OUTER_BOUND('',#17912,.T.);
#11753=FACE_OUTER_BOUND('',#17913,.T.);
#11754=FACE_OUTER_BOUND('',#17914,.T.);
#11755=FACE_OUTER_BOUND('',#17915,.T.);
#11756=FACE_OUTER_BOUND('',#17916,.T.);
#11757=FACE_OUTER_BOUND('',#17917,.T.);
#11758=FACE_OUTER_BOUND('',#17918,.T.);
#11759=FACE_OUTER_BOUND('',#17919,.T.);
#11760=FACE_OUTER_BOUND('',#17920,.T.);
#11761=FACE_OUTER_BOUND('',#17921,.T.);
#11762=FACE_OUTER_BOUND('',#17922,.T.);
#11763=FACE_OUTER_BOUND('',#17923,.T.);
#11764=FACE_OUTER_BOUND('',#17924,.T.);
#11765=FACE_OUTER_BOUND('',#17925,.T.);
#11766=FACE_OUTER_BOUND('',#17926,.T.);
#11767=FACE_OUTER_BOUND('',#17927,.T.);
#11768=FACE_OUTER_BOUND('',#17928,.T.);
#11769=FACE_OUTER_BOUND('',#17929,.T.);
#11770=FACE_OUTER_BOUND('',#17930,.T.);
#11771=FACE_OUTER_BOUND('',#17931,.T.);
#11772=FACE_OUTER_BOUND('',#17932,.T.);
#11773=FACE_OUTER_BOUND('',#17933,.T.);
#11774=FACE_OUTER_BOUND('',#17934,.T.);
#11775=FACE_OUTER_BOUND('',#17935,.T.);
#11776=FACE_OUTER_BOUND('',#17936,.T.);
#11777=FACE_OUTER_BOUND('',#17937,.T.);
#11778=FACE_OUTER_BOUND('',#17938,.T.);
#11779=FACE_OUTER_BOUND('',#17939,.T.);
#11780=FACE_OUTER_BOUND('',#17940,.T.);
#11781=FACE_OUTER_BOUND('',#17941,.T.);
#11782=FACE_OUTER_BOUND('',#17942,.T.);
#11783=FACE_OUTER_BOUND('',#17943,.T.);
#11784=FACE_OUTER_BOUND('',#17944,.T.);
#11785=FACE_OUTER_BOUND('',#17945,.T.);
#11786=FACE_OUTER_BOUND('',#17946,.T.);
#11787=FACE_OUTER_BOUND('',#17947,.T.);
#11788=FACE_OUTER_BOUND('',#17948,.T.);
#11789=FACE_OUTER_BOUND('',#17949,.T.);
#11790=FACE_OUTER_BOUND('',#17950,.T.);
#11791=FACE_OUTER_BOUND('',#17951,.T.);
#11792=FACE_OUTER_BOUND('',#17952,.T.);
#11793=FACE_OUTER_BOUND('',#17953,.T.);
#11794=FACE_OUTER_BOUND('',#17954,.T.);
#11795=FACE_OUTER_BOUND('',#17955,.T.);
#11796=FACE_OUTER_BOUND('',#17956,.T.);
#11797=FACE_OUTER_BOUND('',#17957,.T.);
#11798=FACE_OUTER_BOUND('',#17958,.T.);
#11799=FACE_OUTER_BOUND('',#17959,.T.);
#11800=FACE_OUTER_BOUND('',#17960,.T.);
#11801=FACE_OUTER_BOUND('',#17961,.T.);
#11802=FACE_OUTER_BOUND('',#17962,.T.);
#11803=FACE_OUTER_BOUND('',#17963,.T.);
#11804=FACE_OUTER_BOUND('',#17964,.T.);
#11805=FACE_OUTER_BOUND('',#17965,.T.);
#11806=FACE_OUTER_BOUND('',#17966,.T.);
#11807=FACE_OUTER_BOUND('',#17967,.T.);
#11808=FACE_OUTER_BOUND('',#17968,.T.);
#11809=FACE_OUTER_BOUND('',#17969,.T.);
#11810=FACE_OUTER_BOUND('',#17970,.T.);
#11811=FACE_OUTER_BOUND('',#17971,.T.);
#11812=FACE_OUTER_BOUND('',#17972,.T.);
#11813=FACE_OUTER_BOUND('',#17973,.T.);
#11814=FACE_OUTER_BOUND('',#17974,.T.);
#11815=FACE_OUTER_BOUND('',#17975,.T.);
#11816=FACE_OUTER_BOUND('',#17976,.T.);
#11817=FACE_OUTER_BOUND('',#17977,.T.);
#11818=FACE_OUTER_BOUND('',#17978,.T.);
#11819=FACE_OUTER_BOUND('',#17979,.T.);
#11820=FACE_OUTER_BOUND('',#17980,.T.);
#11821=FACE_OUTER_BOUND('',#17981,.T.);
#11822=FACE_OUTER_BOUND('',#17982,.T.);
#11823=FACE_OUTER_BOUND('',#17983,.T.);
#11824=FACE_OUTER_BOUND('',#17984,.T.);
#11825=FACE_OUTER_BOUND('',#17985,.T.);
#11826=FACE_OUTER_BOUND('',#17986,.T.);
#11827=FACE_OUTER_BOUND('',#17987,.T.);
#11828=FACE_OUTER_BOUND('',#17988,.T.);
#11829=FACE_OUTER_BOUND('',#17989,.T.);
#11830=FACE_OUTER_BOUND('',#17990,.T.);
#11831=FACE_OUTER_BOUND('',#17991,.T.);
#11832=FACE_OUTER_BOUND('',#17992,.T.);
#11833=FACE_OUTER_BOUND('',#17993,.T.);
#11834=FACE_OUTER_BOUND('',#17994,.T.);
#11835=FACE_OUTER_BOUND('',#17995,.T.);
#11836=FACE_OUTER_BOUND('',#17996,.T.);
#11837=FACE_OUTER_BOUND('',#17997,.T.);
#11838=FACE_OUTER_BOUND('',#17998,.T.);
#11839=FACE_OUTER_BOUND('',#17999,.T.);
#11840=FACE_OUTER_BOUND('',#18000,.T.);
#11841=FACE_OUTER_BOUND('',#18001,.T.);
#11842=FACE_OUTER_BOUND('',#18002,.T.);
#11843=FACE_OUTER_BOUND('',#18003,.T.);
#11844=FACE_OUTER_BOUND('',#18004,.T.);
#11845=FACE_OUTER_BOUND('',#18005,.T.);
#11846=FACE_OUTER_BOUND('',#18006,.T.);
#11847=FACE_OUTER_BOUND('',#18007,.T.);
#11848=FACE_OUTER_BOUND('',#18008,.T.);
#11849=FACE_OUTER_BOUND('',#18009,.T.);
#11850=FACE_OUTER_BOUND('',#18010,.T.);
#11851=FACE_OUTER_BOUND('',#18011,.T.);
#11852=FACE_OUTER_BOUND('',#18012,.T.);
#11853=FACE_OUTER_BOUND('',#18013,.T.);
#11854=FACE_OUTER_BOUND('',#18014,.T.);
#11855=FACE_OUTER_BOUND('',#18015,.T.);
#11856=FACE_OUTER_BOUND('',#18016,.T.);
#11857=FACE_OUTER_BOUND('',#18017,.T.);
#11858=FACE_OUTER_BOUND('',#18018,.T.);
#11859=FACE_OUTER_BOUND('',#18019,.T.);
#11860=FACE_OUTER_BOUND('',#18020,.T.);
#11861=FACE_OUTER_BOUND('',#18021,.T.);
#11862=FACE_OUTER_BOUND('',#18022,.T.);
#11863=FACE_OUTER_BOUND('',#18023,.T.);
#11864=FACE_OUTER_BOUND('',#18024,.T.);
#11865=FACE_OUTER_BOUND('',#18025,.T.);
#11866=FACE_OUTER_BOUND('',#18026,.T.);
#11867=FACE_OUTER_BOUND('',#18027,.T.);
#11868=FACE_OUTER_BOUND('',#18028,.T.);
#11869=FACE_OUTER_BOUND('',#18029,.T.);
#11870=FACE_OUTER_BOUND('',#18030,.T.);
#11871=FACE_OUTER_BOUND('',#18031,.T.);
#11872=FACE_OUTER_BOUND('',#18032,.T.);
#11873=FACE_OUTER_BOUND('',#18033,.T.);
#11874=FACE_OUTER_BOUND('',#18034,.T.);
#11875=FACE_OUTER_BOUND('',#18035,.T.);
#11876=FACE_OUTER_BOUND('',#18036,.T.);
#11877=FACE_OUTER_BOUND('',#18037,.T.);
#11878=FACE_OUTER_BOUND('',#18038,.T.);
#11879=FACE_OUTER_BOUND('',#18039,.T.);
#11880=FACE_OUTER_BOUND('',#18040,.T.);
#11881=FACE_OUTER_BOUND('',#18041,.T.);
#11882=FACE_OUTER_BOUND('',#18042,.T.);
#11883=FACE_OUTER_BOUND('',#18043,.T.);
#11884=FACE_OUTER_BOUND('',#18044,.T.);
#11885=FACE_OUTER_BOUND('',#18045,.T.);
#11886=FACE_OUTER_BOUND('',#18046,.T.);
#11887=FACE_OUTER_BOUND('',#18047,.T.);
#11888=FACE_OUTER_BOUND('',#18048,.T.);
#11889=FACE_OUTER_BOUND('',#18049,.T.);
#11890=FACE_OUTER_BOUND('',#18050,.T.);
#11891=FACE_OUTER_BOUND('',#18051,.T.);
#11892=FACE_OUTER_BOUND('',#18052,.T.);
#11893=FACE_OUTER_BOUND('',#18053,.T.);
#11894=FACE_OUTER_BOUND('',#18054,.T.);
#11895=FACE_OUTER_BOUND('',#18055,.T.);
#11896=FACE_OUTER_BOUND('',#18056,.T.);
#11897=FACE_OUTER_BOUND('',#18057,.T.);
#11898=FACE_OUTER_BOUND('',#18058,.T.);
#11899=FACE_OUTER_BOUND('',#18059,.T.);
#11900=FACE_OUTER_BOUND('',#18060,.T.);
#11901=FACE_OUTER_BOUND('',#18061,.T.);
#11902=FACE_OUTER_BOUND('',#18062,.T.);
#11903=FACE_OUTER_BOUND('',#18063,.T.);
#11904=FACE_OUTER_BOUND('',#18064,.T.);
#11905=FACE_OUTER_BOUND('',#18065,.T.);
#11906=FACE_OUTER_BOUND('',#18066,.T.);
#11907=FACE_OUTER_BOUND('',#18067,.T.);
#11908=FACE_OUTER_BOUND('',#18068,.T.);
#11909=FACE_OUTER_BOUND('',#18069,.T.);
#11910=FACE_OUTER_BOUND('',#18070,.T.);
#11911=FACE_OUTER_BOUND('',#18071,.T.);
#11912=FACE_OUTER_BOUND('',#18072,.T.);
#11913=FACE_OUTER_BOUND('',#18073,.T.);
#11914=FACE_OUTER_BOUND('',#18074,.T.);
#11915=FACE_OUTER_BOUND('',#18075,.T.);
#11916=FACE_OUTER_BOUND('',#18076,.T.);
#11917=FACE_OUTER_BOUND('',#18077,.T.);
#11918=FACE_OUTER_BOUND('',#18078,.T.);
#11919=FACE_OUTER_BOUND('',#18079,.T.);
#11920=FACE_OUTER_BOUND('',#18080,.T.);
#11921=FACE_OUTER_BOUND('',#18081,.T.);
#11922=FACE_OUTER_BOUND('',#18082,.T.);
#11923=FACE_OUTER_BOUND('',#18083,.T.);
#11924=FACE_OUTER_BOUND('',#18084,.T.);
#11925=FACE_OUTER_BOUND('',#18085,.T.);
#11926=FACE_OUTER_BOUND('',#18086,.T.);
#11927=FACE_OUTER_BOUND('',#18087,.T.);
#11928=FACE_OUTER_BOUND('',#18088,.T.);
#11929=FACE_OUTER_BOUND('',#18089,.T.);
#11930=FACE_OUTER_BOUND('',#18090,.T.);
#11931=FACE_OUTER_BOUND('',#18091,.T.);
#11932=FACE_OUTER_BOUND('',#18092,.T.);
#11933=FACE_OUTER_BOUND('',#18093,.T.);
#11934=FACE_OUTER_BOUND('',#18094,.T.);
#11935=FACE_OUTER_BOUND('',#18095,.T.);
#11936=FACE_OUTER_BOUND('',#18096,.T.);
#11937=FACE_OUTER_BOUND('',#18097,.T.);
#11938=FACE_OUTER_BOUND('',#18098,.T.);
#11939=FACE_OUTER_BOUND('',#18099,.T.);
#11940=FACE_OUTER_BOUND('',#18100,.T.);
#11941=FACE_OUTER_BOUND('',#18101,.T.);
#11942=FACE_OUTER_BOUND('',#18102,.T.);
#11943=FACE_OUTER_BOUND('',#18103,.T.);
#11944=FACE_OUTER_BOUND('',#18104,.T.);
#11945=FACE_OUTER_BOUND('',#18105,.T.);
#11946=FACE_OUTER_BOUND('',#18106,.T.);
#11947=FACE_OUTER_BOUND('',#18107,.T.);
#11948=FACE_OUTER_BOUND('',#18108,.T.);
#11949=FACE_OUTER_BOUND('',#18109,.T.);
#11950=FACE_OUTER_BOUND('',#18110,.T.);
#11951=FACE_OUTER_BOUND('',#18111,.T.);
#11952=FACE_OUTER_BOUND('',#18112,.T.);
#11953=FACE_OUTER_BOUND('',#18113,.T.);
#11954=FACE_OUTER_BOUND('',#18114,.T.);
#11955=FACE_OUTER_BOUND('',#18115,.T.);
#11956=FACE_OUTER_BOUND('',#18116,.T.);
#11957=FACE_OUTER_BOUND('',#18117,.T.);
#11958=FACE_OUTER_BOUND('',#18118,.T.);
#11959=FACE_OUTER_BOUND('',#18119,.T.);
#11960=FACE_OUTER_BOUND('',#18120,.T.);
#11961=FACE_OUTER_BOUND('',#18121,.T.);
#11962=FACE_OUTER_BOUND('',#18122,.T.);
#11963=FACE_OUTER_BOUND('',#18123,.T.);
#11964=FACE_OUTER_BOUND('',#18124,.T.);
#11965=FACE_OUTER_BOUND('',#18125,.T.);
#11966=FACE_OUTER_BOUND('',#18126,.T.);
#11967=FACE_OUTER_BOUND('',#18127,.T.);
#11968=FACE_OUTER_BOUND('',#18128,.T.);
#11969=FACE_OUTER_BOUND('',#18129,.T.);
#11970=FACE_OUTER_BOUND('',#18130,.T.);
#11971=FACE_OUTER_BOUND('',#18131,.T.);
#11972=FACE_OUTER_BOUND('',#18132,.T.);
#11973=FACE_OUTER_BOUND('',#18133,.T.);
#11974=FACE_OUTER_BOUND('',#18134,.T.);
#11975=FACE_OUTER_BOUND('',#18135,.T.);
#11976=FACE_OUTER_BOUND('',#18136,.T.);
#11977=FACE_OUTER_BOUND('',#18137,.T.);
#11978=FACE_OUTER_BOUND('',#18138,.T.);
#11979=FACE_OUTER_BOUND('',#18139,.T.);
#11980=FACE_OUTER_BOUND('',#18140,.T.);
#11981=FACE_OUTER_BOUND('',#18141,.T.);
#11982=FACE_OUTER_BOUND('',#18142,.T.);
#11983=FACE_OUTER_BOUND('',#18143,.T.);
#11984=FACE_OUTER_BOUND('',#18144,.T.);
#11985=FACE_OUTER_BOUND('',#18145,.T.);
#11986=FACE_OUTER_BOUND('',#18146,.T.);
#11987=FACE_OUTER_BOUND('',#18147,.T.);
#11988=FACE_OUTER_BOUND('',#18148,.T.);
#11989=FACE_OUTER_BOUND('',#18149,.T.);
#11990=FACE_OUTER_BOUND('',#18150,.T.);
#11991=FACE_OUTER_BOUND('',#18151,.T.);
#11992=FACE_OUTER_BOUND('',#18152,.T.);
#11993=FACE_OUTER_BOUND('',#18153,.T.);
#11994=FACE_OUTER_BOUND('',#18154,.T.);
#11995=FACE_OUTER_BOUND('',#18155,.T.);
#11996=FACE_OUTER_BOUND('',#18156,.T.);
#11997=FACE_OUTER_BOUND('',#18157,.T.);
#11998=FACE_OUTER_BOUND('',#18158,.T.);
#11999=FACE_OUTER_BOUND('',#18159,.T.);
#12000=FACE_OUTER_BOUND('',#18160,.T.);
#12001=FACE_OUTER_BOUND('',#18161,.T.);
#12002=FACE_OUTER_BOUND('',#18162,.T.);
#12003=FACE_OUTER_BOUND('',#18163,.T.);
#12004=FACE_OUTER_BOUND('',#18164,.T.);
#12005=FACE_OUTER_BOUND('',#18165,.T.);
#12006=FACE_OUTER_BOUND('',#18166,.T.);
#12007=FACE_OUTER_BOUND('',#18167,.T.);
#12008=FACE_OUTER_BOUND('',#18168,.T.);
#12009=FACE_OUTER_BOUND('',#18169,.T.);
#12010=FACE_OUTER_BOUND('',#18170,.T.);
#12011=FACE_OUTER_BOUND('',#18171,.T.);
#12012=FACE_OUTER_BOUND('',#18172,.T.);
#12013=FACE_OUTER_BOUND('',#18173,.T.);
#12014=FACE_OUTER_BOUND('',#18174,.T.);
#12015=FACE_OUTER_BOUND('',#18175,.T.);
#12016=FACE_OUTER_BOUND('',#18176,.T.);
#12017=FACE_OUTER_BOUND('',#18177,.T.);
#12018=FACE_OUTER_BOUND('',#18178,.T.);
#12019=FACE_OUTER_BOUND('',#18179,.T.);
#12020=FACE_OUTER_BOUND('',#18180,.T.);
#12021=FACE_OUTER_BOUND('',#18181,.T.);
#12022=FACE_OUTER_BOUND('',#18182,.T.);
#12023=FACE_OUTER_BOUND('',#18183,.T.);
#12024=FACE_OUTER_BOUND('',#18184,.T.);
#12025=FACE_OUTER_BOUND('',#18185,.T.);
#12026=FACE_OUTER_BOUND('',#18186,.T.);
#12027=FACE_OUTER_BOUND('',#18187,.T.);
#12028=FACE_OUTER_BOUND('',#18188,.T.);
#12029=FACE_OUTER_BOUND('',#18189,.T.);
#12030=FACE_OUTER_BOUND('',#18190,.T.);
#12031=FACE_OUTER_BOUND('',#18191,.T.);
#12032=FACE_OUTER_BOUND('',#18192,.T.);
#12033=FACE_OUTER_BOUND('',#18193,.T.);
#12034=FACE_OUTER_BOUND('',#18194,.T.);
#12035=FACE_OUTER_BOUND('',#18195,.T.);
#12036=FACE_OUTER_BOUND('',#18196,.T.);
#12037=FACE_OUTER_BOUND('',#18197,.T.);
#12038=FACE_OUTER_BOUND('',#18198,.T.);
#12039=FACE_OUTER_BOUND('',#18199,.T.);
#12040=FACE_OUTER_BOUND('',#18200,.T.);
#12041=FACE_OUTER_BOUND('',#18201,.T.);
#12042=FACE_OUTER_BOUND('',#18202,.T.);
#12043=FACE_OUTER_BOUND('',#18203,.T.);
#12044=FACE_OUTER_BOUND('',#18204,.T.);
#12045=FACE_OUTER_BOUND('',#18205,.T.);
#12046=FACE_OUTER_BOUND('',#18206,.T.);
#12047=FACE_OUTER_BOUND('',#18207,.T.);
#12048=FACE_OUTER_BOUND('',#18208,.T.);
#12049=FACE_OUTER_BOUND('',#18209,.T.);
#12050=FACE_OUTER_BOUND('',#18210,.T.);
#12051=FACE_OUTER_BOUND('',#18211,.T.);
#12052=FACE_OUTER_BOUND('',#18212,.T.);
#12053=FACE_OUTER_BOUND('',#18213,.T.);
#12054=FACE_OUTER_BOUND('',#18214,.T.);
#12055=FACE_OUTER_BOUND('',#18215,.T.);
#12056=FACE_OUTER_BOUND('',#18216,.T.);
#12057=FACE_OUTER_BOUND('',#18217,.T.);
#12058=FACE_OUTER_BOUND('',#18218,.T.);
#12059=FACE_OUTER_BOUND('',#18219,.T.);
#12060=FACE_OUTER_BOUND('',#18220,.T.);
#12061=FACE_OUTER_BOUND('',#18221,.T.);
#12062=FACE_OUTER_BOUND('',#18222,.T.);
#12063=FACE_OUTER_BOUND('',#18223,.T.);
#12064=FACE_OUTER_BOUND('',#18224,.T.);
#12065=FACE_OUTER_BOUND('',#18225,.T.);
#12066=FACE_OUTER_BOUND('',#18226,.T.);
#12067=FACE_OUTER_BOUND('',#18227,.T.);
#12068=FACE_OUTER_BOUND('',#18228,.T.);
#12069=FACE_OUTER_BOUND('',#18229,.T.);
#12070=FACE_OUTER_BOUND('',#18230,.T.);
#12071=FACE_OUTER_BOUND('',#18231,.T.);
#12072=FACE_OUTER_BOUND('',#18232,.T.);
#12073=FACE_OUTER_BOUND('',#18233,.T.);
#12074=FACE_OUTER_BOUND('',#18234,.T.);
#12075=FACE_OUTER_BOUND('',#18235,.T.);
#12076=FACE_OUTER_BOUND('',#18236,.T.);
#12077=FACE_OUTER_BOUND('',#18237,.T.);
#12078=FACE_OUTER_BOUND('',#18238,.T.);
#12079=FACE_OUTER_BOUND('',#18239,.T.);
#12080=FACE_OUTER_BOUND('',#18240,.T.);
#12081=FACE_OUTER_BOUND('',#18241,.T.);
#12082=FACE_OUTER_BOUND('',#18242,.T.);
#12083=FACE_OUTER_BOUND('',#18243,.T.);
#12084=FACE_OUTER_BOUND('',#18244,.T.);
#12085=FACE_OUTER_BOUND('',#18245,.T.);
#12086=FACE_OUTER_BOUND('',#18246,.T.);
#12087=FACE_OUTER_BOUND('',#18247,.T.);
#12088=FACE_OUTER_BOUND('',#18248,.T.);
#12089=FACE_OUTER_BOUND('',#18249,.T.);
#12090=FACE_OUTER_BOUND('',#18250,.T.);
#12091=FACE_OUTER_BOUND('',#18251,.T.);
#12092=FACE_OUTER_BOUND('',#18252,.T.);
#12093=FACE_OUTER_BOUND('',#18253,.T.);
#12094=FACE_OUTER_BOUND('',#18254,.T.);
#12095=FACE_OUTER_BOUND('',#18255,.T.);
#12096=FACE_OUTER_BOUND('',#18256,.T.);
#12097=FACE_OUTER_BOUND('',#18257,.T.);
#12098=FACE_OUTER_BOUND('',#18258,.T.);
#12099=FACE_OUTER_BOUND('',#18259,.T.);
#12100=FACE_OUTER_BOUND('',#18260,.T.);
#12101=FACE_OUTER_BOUND('',#18261,.T.);
#12102=FACE_OUTER_BOUND('',#18262,.T.);
#12103=FACE_OUTER_BOUND('',#18263,.T.);
#12104=FACE_OUTER_BOUND('',#18264,.T.);
#12105=FACE_OUTER_BOUND('',#18265,.T.);
#12106=FACE_OUTER_BOUND('',#18266,.T.);
#12107=FACE_OUTER_BOUND('',#18267,.T.);
#12108=FACE_OUTER_BOUND('',#18268,.T.);
#12109=FACE_OUTER_BOUND('',#18269,.T.);
#12110=FACE_OUTER_BOUND('',#18270,.T.);
#12111=FACE_OUTER_BOUND('',#18271,.T.);
#12112=FACE_OUTER_BOUND('',#18272,.T.);
#12113=FACE_OUTER_BOUND('',#18273,.T.);
#12114=FACE_OUTER_BOUND('',#18274,.T.);
#12115=FACE_OUTER_BOUND('',#18275,.T.);
#12116=FACE_OUTER_BOUND('',#18276,.T.);
#12117=FACE_OUTER_BOUND('',#18277,.T.);
#12118=FACE_OUTER_BOUND('',#18278,.T.);
#12119=FACE_OUTER_BOUND('',#18279,.T.);
#12120=FACE_OUTER_BOUND('',#18280,.T.);
#12121=FACE_OUTER_BOUND('',#18281,.T.);
#12122=FACE_OUTER_BOUND('',#18282,.T.);
#12123=FACE_OUTER_BOUND('',#18283,.T.);
#12124=FACE_OUTER_BOUND('',#18284,.T.);
#12125=FACE_OUTER_BOUND('',#18285,.T.);
#12126=FACE_OUTER_BOUND('',#18286,.T.);
#12127=FACE_OUTER_BOUND('',#18287,.T.);
#12128=FACE_OUTER_BOUND('',#18288,.T.);
#12129=FACE_OUTER_BOUND('',#18289,.T.);
#12130=FACE_OUTER_BOUND('',#18290,.T.);
#12131=FACE_OUTER_BOUND('',#18291,.T.);
#12132=FACE_OUTER_BOUND('',#18292,.T.);
#12133=FACE_OUTER_BOUND('',#18293,.T.);
#12134=FACE_OUTER_BOUND('',#18294,.T.);
#12135=FACE_OUTER_BOUND('',#18295,.T.);
#12136=FACE_OUTER_BOUND('',#18296,.T.);
#12137=FACE_OUTER_BOUND('',#18297,.T.);
#12138=FACE_OUTER_BOUND('',#18298,.T.);
#12139=FACE_OUTER_BOUND('',#18299,.T.);
#12140=FACE_OUTER_BOUND('',#18300,.T.);
#12141=FACE_OUTER_BOUND('',#18301,.T.);
#12142=FACE_OUTER_BOUND('',#18302,.T.);
#12143=FACE_OUTER_BOUND('',#18303,.T.);
#12144=FACE_OUTER_BOUND('',#18304,.T.);
#12145=FACE_OUTER_BOUND('',#18305,.T.);
#12146=FACE_OUTER_BOUND('',#18306,.T.);
#12147=FACE_OUTER_BOUND('',#18307,.T.);
#12148=FACE_OUTER_BOUND('',#18308,.T.);
#12149=FACE_OUTER_BOUND('',#18309,.T.);
#12150=FACE_OUTER_BOUND('',#18310,.T.);
#12151=FACE_OUTER_BOUND('',#18311,.T.);
#12152=FACE_OUTER_BOUND('',#18312,.T.);
#12153=FACE_OUTER_BOUND('',#18313,.T.);
#12154=FACE_OUTER_BOUND('',#18314,.T.);
#12155=FACE_OUTER_BOUND('',#18315,.T.);
#12156=FACE_OUTER_BOUND('',#18316,.T.);
#12157=FACE_OUTER_BOUND('',#18317,.T.);
#12158=FACE_OUTER_BOUND('',#18318,.T.);
#12159=FACE_OUTER_BOUND('',#18319,.T.);
#12160=FACE_OUTER_BOUND('',#18320,.T.);
#12161=FACE_OUTER_BOUND('',#18321,.T.);
#12162=FACE_OUTER_BOUND('',#18322,.T.);
#12163=FACE_OUTER_BOUND('',#18323,.T.);
#12164=FACE_OUTER_BOUND('',#18324,.T.);
#12165=FACE_OUTER_BOUND('',#18325,.T.);
#12166=FACE_OUTER_BOUND('',#18326,.T.);
#12167=FACE_OUTER_BOUND('',#18327,.T.);
#12168=FACE_OUTER_BOUND('',#18328,.T.);
#12169=FACE_OUTER_BOUND('',#18329,.T.);
#12170=FACE_OUTER_BOUND('',#18330,.T.);
#12171=FACE_OUTER_BOUND('',#18331,.T.);
#12172=FACE_OUTER_BOUND('',#18332,.T.);
#12173=FACE_OUTER_BOUND('',#18333,.T.);
#12174=FACE_OUTER_BOUND('',#18334,.T.);
#12175=FACE_OUTER_BOUND('',#18335,.T.);
#12176=FACE_OUTER_BOUND('',#18336,.T.);
#12177=FACE_OUTER_BOUND('',#18337,.T.);
#12178=FACE_OUTER_BOUND('',#18338,.T.);
#12179=FACE_OUTER_BOUND('',#18339,.T.);
#12180=FACE_OUTER_BOUND('',#18340,.T.);
#12181=FACE_OUTER_BOUND('',#18341,.T.);
#12182=FACE_OUTER_BOUND('',#18342,.T.);
#12183=FACE_OUTER_BOUND('',#18343,.T.);
#12184=FACE_OUTER_BOUND('',#18344,.T.);
#12185=FACE_OUTER_BOUND('',#18345,.T.);
#12186=FACE_OUTER_BOUND('',#18346,.T.);
#12187=FACE_OUTER_BOUND('',#18347,.T.);
#12188=FACE_OUTER_BOUND('',#18348,.T.);
#12189=FACE_OUTER_BOUND('',#18349,.T.);
#12190=FACE_OUTER_BOUND('',#18350,.T.);
#12191=FACE_OUTER_BOUND('',#18351,.T.);
#12192=FACE_OUTER_BOUND('',#18352,.T.);
#12193=FACE_OUTER_BOUND('',#18353,.T.);
#12194=FACE_OUTER_BOUND('',#18354,.T.);
#12195=FACE_OUTER_BOUND('',#18355,.T.);
#12196=FACE_OUTER_BOUND('',#18356,.T.);
#12197=FACE_OUTER_BOUND('',#18357,.T.);
#12198=FACE_OUTER_BOUND('',#18358,.T.);
#12199=FACE_OUTER_BOUND('',#18359,.T.);
#12200=FACE_OUTER_BOUND('',#18360,.T.);
#12201=FACE_OUTER_BOUND('',#18361,.T.);
#12202=FACE_OUTER_BOUND('',#18362,.T.);
#12203=FACE_OUTER_BOUND('',#18363,.T.);
#12204=FACE_OUTER_BOUND('',#18364,.T.);
#12205=FACE_OUTER_BOUND('',#18365,.T.);
#12206=FACE_OUTER_BOUND('',#18366,.T.);
#12207=FACE_OUTER_BOUND('',#18367,.T.);
#12208=FACE_OUTER_BOUND('',#18368,.T.);
#12209=FACE_OUTER_BOUND('',#18369,.T.);
#12210=FACE_OUTER_BOUND('',#18370,.T.);
#12211=FACE_OUTER_BOUND('',#18371,.T.);
#12212=FACE_OUTER_BOUND('',#18372,.T.);
#12213=FACE_OUTER_BOUND('',#18373,.T.);
#12214=FACE_OUTER_BOUND('',#18374,.T.);
#12215=FACE_OUTER_BOUND('',#18375,.T.);
#12216=FACE_OUTER_BOUND('',#18376,.T.);
#12217=FACE_OUTER_BOUND('',#18377,.T.);
#12218=FACE_OUTER_BOUND('',#18378,.T.);
#12219=FACE_OUTER_BOUND('',#18379,.T.);
#12220=FACE_OUTER_BOUND('',#18380,.T.);
#12221=FACE_OUTER_BOUND('',#18381,.T.);
#12222=FACE_OUTER_BOUND('',#18382,.T.);
#12223=FACE_OUTER_BOUND('',#18383,.T.);
#12224=FACE_OUTER_BOUND('',#18384,.T.);
#12225=FACE_OUTER_BOUND('',#18385,.T.);
#12226=FACE_OUTER_BOUND('',#18386,.T.);
#12227=FACE_OUTER_BOUND('',#18387,.T.);
#12228=FACE_OUTER_BOUND('',#18388,.T.);
#12229=FACE_OUTER_BOUND('',#18389,.T.);
#12230=FACE_OUTER_BOUND('',#18390,.T.);
#12231=FACE_OUTER_BOUND('',#18391,.T.);
#12232=FACE_OUTER_BOUND('',#18392,.T.);
#12233=FACE_OUTER_BOUND('',#18393,.T.);
#12234=FACE_OUTER_BOUND('',#18394,.T.);
#12235=FACE_OUTER_BOUND('',#18395,.T.);
#12236=FACE_OUTER_BOUND('',#18396,.T.);
#12237=FACE_OUTER_BOUND('',#18397,.T.);
#12238=FACE_OUTER_BOUND('',#18398,.T.);
#12239=FACE_OUTER_BOUND('',#18399,.T.);
#12240=FACE_OUTER_BOUND('',#18400,.T.);
#12241=FACE_OUTER_BOUND('',#18401,.T.);
#12242=FACE_OUTER_BOUND('',#18402,.T.);
#12243=FACE_OUTER_BOUND('',#18403,.T.);
#12244=FACE_OUTER_BOUND('',#18404,.T.);
#12245=FACE_OUTER_BOUND('',#18405,.T.);
#12246=FACE_OUTER_BOUND('',#18406,.T.);
#12247=FACE_OUTER_BOUND('',#18407,.T.);
#12248=FACE_OUTER_BOUND('',#18408,.T.);
#12249=FACE_OUTER_BOUND('',#18409,.T.);
#12250=FACE_OUTER_BOUND('',#18410,.T.);
#12251=FACE_OUTER_BOUND('',#18411,.T.);
#12252=FACE_OUTER_BOUND('',#18412,.T.);
#12253=FACE_OUTER_BOUND('',#18413,.T.);
#12254=FACE_OUTER_BOUND('',#18414,.T.);
#12255=FACE_OUTER_BOUND('',#18415,.T.);
#12256=FACE_OUTER_BOUND('',#18416,.T.);
#12257=FACE_OUTER_BOUND('',#18417,.T.);
#12258=FACE_OUTER_BOUND('',#18418,.T.);
#12259=FACE_OUTER_BOUND('',#18419,.T.);
#12260=FACE_OUTER_BOUND('',#18420,.T.);
#12261=FACE_OUTER_BOUND('',#18421,.T.);
#12262=FACE_OUTER_BOUND('',#18422,.T.);
#12263=FACE_OUTER_BOUND('',#18423,.T.);
#12264=FACE_OUTER_BOUND('',#18424,.T.);
#12265=FACE_OUTER_BOUND('',#18425,.T.);
#12266=FACE_OUTER_BOUND('',#18426,.T.);
#12267=FACE_OUTER_BOUND('',#18427,.T.);
#12268=FACE_OUTER_BOUND('',#18428,.T.);
#12269=FACE_OUTER_BOUND('',#18429,.T.);
#12270=FACE_OUTER_BOUND('',#18430,.T.);
#12271=FACE_OUTER_BOUND('',#18431,.T.);
#12272=FACE_OUTER_BOUND('',#18432,.T.);
#12273=FACE_OUTER_BOUND('',#18433,.T.);
#12274=FACE_OUTER_BOUND('',#18434,.T.);
#12275=FACE_OUTER_BOUND('',#18435,.T.);
#12276=FACE_OUTER_BOUND('',#18436,.T.);
#12277=FACE_OUTER_BOUND('',#18437,.T.);
#12278=FACE_OUTER_BOUND('',#18438,.T.);
#12279=FACE_OUTER_BOUND('',#18439,.T.);
#12280=FACE_OUTER_BOUND('',#18440,.T.);
#12281=FACE_OUTER_BOUND('',#18441,.T.);
#12282=FACE_OUTER_BOUND('',#18442,.T.);
#12283=FACE_OUTER_BOUND('',#18443,.T.);
#12284=FACE_OUTER_BOUND('',#18444,.T.);
#12285=FACE_OUTER_BOUND('',#18445,.T.);
#12286=FACE_OUTER_BOUND('',#18446,.T.);
#12287=FACE_OUTER_BOUND('',#18447,.T.);
#12288=FACE_OUTER_BOUND('',#18448,.T.);
#12289=FACE_OUTER_BOUND('',#18449,.T.);
#12290=FACE_OUTER_BOUND('',#18450,.T.);
#12291=FACE_OUTER_BOUND('',#18451,.T.);
#12292=FACE_OUTER_BOUND('',#18452,.T.);
#12293=FACE_OUTER_BOUND('',#18453,.T.);
#12294=FACE_OUTER_BOUND('',#18454,.T.);
#12295=FACE_OUTER_BOUND('',#18455,.T.);
#12296=FACE_OUTER_BOUND('',#18456,.T.);
#12297=FACE_OUTER_BOUND('',#18457,.T.);
#12298=FACE_OUTER_BOUND('',#18458,.T.);
#12299=FACE_OUTER_BOUND('',#18459,.T.);
#12300=FACE_OUTER_BOUND('',#18460,.T.);
#12301=FACE_OUTER_BOUND('',#18461,.T.);
#12302=FACE_OUTER_BOUND('',#18462,.T.);
#12303=FACE_OUTER_BOUND('',#18463,.T.);
#12304=FACE_OUTER_BOUND('',#18464,.T.);
#12305=FACE_OUTER_BOUND('',#18465,.T.);
#12306=FACE_OUTER_BOUND('',#18466,.T.);
#12307=FACE_OUTER_BOUND('',#18467,.T.);
#12308=FACE_OUTER_BOUND('',#18468,.T.);
#12309=FACE_OUTER_BOUND('',#18469,.T.);
#12310=FACE_OUTER_BOUND('',#18470,.T.);
#12311=FACE_OUTER_BOUND('',#18471,.T.);
#12312=FACE_OUTER_BOUND('',#18472,.T.);
#12313=FACE_OUTER_BOUND('',#18473,.T.);
#12314=FACE_OUTER_BOUND('',#18474,.T.);
#12315=FACE_OUTER_BOUND('',#18475,.T.);
#12316=FACE_OUTER_BOUND('',#18476,.T.);
#12317=FACE_OUTER_BOUND('',#18477,.T.);
#12318=FACE_OUTER_BOUND('',#18478,.T.);
#12319=FACE_OUTER_BOUND('',#18479,.T.);
#12320=FACE_OUTER_BOUND('',#18480,.T.);
#12321=FACE_OUTER_BOUND('',#18481,.T.);
#12322=FACE_OUTER_BOUND('',#18482,.T.);
#12323=FACE_OUTER_BOUND('',#18483,.T.);
#12324=FACE_OUTER_BOUND('',#18484,.T.);
#12325=FACE_OUTER_BOUND('',#18485,.T.);
#12326=FACE_OUTER_BOUND('',#18486,.T.);
#12327=FACE_OUTER_BOUND('',#18487,.T.);
#12328=FACE_OUTER_BOUND('',#18488,.T.);
#12329=FACE_OUTER_BOUND('',#18489,.T.);
#12330=FACE_OUTER_BOUND('',#18490,.T.);
#12331=FACE_OUTER_BOUND('',#18491,.T.);
#12332=FACE_OUTER_BOUND('',#18492,.T.);
#12333=FACE_OUTER_BOUND('',#18493,.T.);
#12334=FACE_OUTER_BOUND('',#18494,.T.);
#12335=FACE_OUTER_BOUND('',#18495,.T.);
#12336=FACE_OUTER_BOUND('',#18496,.T.);
#12337=FACE_OUTER_BOUND('',#18497,.T.);
#12338=FACE_OUTER_BOUND('',#18498,.T.);
#12339=FACE_OUTER_BOUND('',#18499,.T.);
#12340=FACE_OUTER_BOUND('',#18500,.T.);
#12341=FACE_OUTER_BOUND('',#18501,.T.);
#12342=FACE_OUTER_BOUND('',#18502,.T.);
#12343=FACE_OUTER_BOUND('',#18503,.T.);
#12344=FACE_OUTER_BOUND('',#18504,.T.);
#12345=FACE_OUTER_BOUND('',#18505,.T.);
#12346=FACE_OUTER_BOUND('',#18506,.T.);
#12347=FACE_OUTER_BOUND('',#18507,.T.);
#12348=FACE_OUTER_BOUND('',#18508,.T.);
#12349=FACE_OUTER_BOUND('',#18509,.T.);
#12350=FACE_OUTER_BOUND('',#18510,.T.);
#12351=FACE_OUTER_BOUND('',#18511,.T.);
#12352=FACE_OUTER_BOUND('',#18512,.T.);
#12353=FACE_OUTER_BOUND('',#18513,.T.);
#12354=FACE_OUTER_BOUND('',#18514,.T.);
#12355=FACE_OUTER_BOUND('',#18515,.T.);
#12356=FACE_OUTER_BOUND('',#18516,.T.);
#12357=FACE_OUTER_BOUND('',#18517,.T.);
#12358=FACE_OUTER_BOUND('',#18518,.T.);
#12359=FACE_OUTER_BOUND('',#18519,.T.);
#12360=FACE_OUTER_BOUND('',#18520,.T.);
#12361=FACE_OUTER_BOUND('',#18521,.T.);
#12362=FACE_OUTER_BOUND('',#18522,.T.);
#12363=FACE_OUTER_BOUND('',#18523,.T.);
#12364=FACE_OUTER_BOUND('',#18524,.T.);
#12365=FACE_OUTER_BOUND('',#18525,.T.);
#12366=FACE_OUTER_BOUND('',#18526,.T.);
#12367=FACE_OUTER_BOUND('',#18527,.T.);
#12368=FACE_OUTER_BOUND('',#18528,.T.);
#12369=FACE_OUTER_BOUND('',#18529,.T.);
#12370=FACE_OUTER_BOUND('',#18530,.T.);
#12371=FACE_OUTER_BOUND('',#18531,.T.);
#12372=FACE_OUTER_BOUND('',#18532,.T.);
#12373=FACE_OUTER_BOUND('',#18533,.T.);
#12374=FACE_OUTER_BOUND('',#18534,.T.);
#12375=FACE_OUTER_BOUND('',#18535,.T.);
#12376=FACE_OUTER_BOUND('',#18536,.T.);
#12377=FACE_OUTER_BOUND('',#18537,.T.);
#12378=FACE_OUTER_BOUND('',#18538,.T.);
#12379=FACE_OUTER_BOUND('',#18539,.T.);
#12380=FACE_OUTER_BOUND('',#18540,.T.);
#12381=FACE_OUTER_BOUND('',#18541,.T.);
#12382=FACE_OUTER_BOUND('',#18542,.T.);
#12383=FACE_OUTER_BOUND('',#18543,.T.);
#12384=FACE_OUTER_BOUND('',#18544,.T.);
#12385=FACE_OUTER_BOUND('',#18545,.T.);
#12386=FACE_OUTER_BOUND('',#18546,.T.);
#12387=FACE_OUTER_BOUND('',#18547,.T.);
#12388=FACE_OUTER_BOUND('',#18548,.T.);
#12389=FACE_OUTER_BOUND('',#18549,.T.);
#12390=FACE_OUTER_BOUND('',#18550,.T.);
#12391=FACE_OUTER_BOUND('',#18551,.T.);
#12392=FACE_OUTER_BOUND('',#18552,.T.);
#12393=FACE_OUTER_BOUND('',#18553,.T.);
#12394=FACE_OUTER_BOUND('',#18554,.T.);
#12395=FACE_OUTER_BOUND('',#18555,.T.);
#12396=FACE_OUTER_BOUND('',#18556,.T.);
#12397=FACE_OUTER_BOUND('',#18557,.T.);
#12398=FACE_OUTER_BOUND('',#18558,.T.);
#12399=FACE_OUTER_BOUND('',#18559,.T.);
#12400=FACE_OUTER_BOUND('',#18560,.T.);
#12401=FACE_OUTER_BOUND('',#18561,.T.);
#12402=FACE_OUTER_BOUND('',#18562,.T.);
#12403=FACE_OUTER_BOUND('',#18563,.T.);
#12404=FACE_OUTER_BOUND('',#18564,.T.);
#12405=FACE_OUTER_BOUND('',#18565,.T.);
#12406=FACE_OUTER_BOUND('',#18566,.T.);
#12407=FACE_OUTER_BOUND('',#18567,.T.);
#12408=FACE_OUTER_BOUND('',#18568,.T.);
#12409=FACE_OUTER_BOUND('',#18569,.T.);
#12410=FACE_OUTER_BOUND('',#18570,.T.);
#12411=FACE_OUTER_BOUND('',#18571,.T.);
#12412=FACE_OUTER_BOUND('',#18572,.T.);
#12413=FACE_OUTER_BOUND('',#18573,.T.);
#12414=FACE_OUTER_BOUND('',#18574,.T.);
#12415=FACE_OUTER_BOUND('',#18575,.T.);
#12416=FACE_OUTER_BOUND('',#18576,.T.);
#12417=FACE_OUTER_BOUND('',#18577,.T.);
#12418=FACE_OUTER_BOUND('',#18578,.T.);
#12419=FACE_OUTER_BOUND('',#18579,.T.);
#12420=FACE_OUTER_BOUND('',#18580,.T.);
#12421=FACE_OUTER_BOUND('',#18581,.T.);
#12422=FACE_OUTER_BOUND('',#18582,.T.);
#12423=FACE_OUTER_BOUND('',#18583,.T.);
#12424=FACE_OUTER_BOUND('',#18584,.T.);
#12425=FACE_OUTER_BOUND('',#18585,.T.);
#12426=FACE_OUTER_BOUND('',#18586,.T.);
#12427=FACE_OUTER_BOUND('',#18587,.T.);
#12428=FACE_OUTER_BOUND('',#18588,.T.);
#12429=FACE_OUTER_BOUND('',#18589,.T.);
#12430=FACE_OUTER_BOUND('',#18590,.T.);
#12431=FACE_OUTER_BOUND('',#18591,.T.);
#12432=FACE_OUTER_BOUND('',#18592,.T.);
#12433=FACE_OUTER_BOUND('',#18593,.T.);
#12434=FACE_OUTER_BOUND('',#18594,.T.);
#12435=FACE_OUTER_BOUND('',#18595,.T.);
#12436=FACE_OUTER_BOUND('',#18596,.T.);
#12437=FACE_OUTER_BOUND('',#18597,.T.);
#12438=FACE_OUTER_BOUND('',#18598,.T.);
#12439=FACE_OUTER_BOUND('',#18599,.T.);
#12440=FACE_OUTER_BOUND('',#18600,.T.);
#12441=FACE_OUTER_BOUND('',#18601,.T.);
#12442=FACE_OUTER_BOUND('',#18602,.T.);
#12443=FACE_OUTER_BOUND('',#18603,.T.);
#12444=FACE_OUTER_BOUND('',#18604,.T.);
#12445=FACE_OUTER_BOUND('',#18605,.T.);
#12446=FACE_OUTER_BOUND('',#18606,.T.);
#12447=FACE_OUTER_BOUND('',#18607,.T.);
#12448=FACE_OUTER_BOUND('',#18608,.T.);
#12449=FACE_OUTER_BOUND('',#18609,.T.);
#12450=FACE_OUTER_BOUND('',#18610,.T.);
#12451=FACE_OUTER_BOUND('',#18611,.T.);
#12452=FACE_OUTER_BOUND('',#18612,.T.);
#12453=FACE_OUTER_BOUND('',#18613,.T.);
#12454=FACE_OUTER_BOUND('',#18614,.T.);
#12455=FACE_OUTER_BOUND('',#18615,.T.);
#12456=FACE_OUTER_BOUND('',#18616,.T.);
#12457=FACE_OUTER_BOUND('',#18617,.T.);
#12458=FACE_OUTER_BOUND('',#18618,.T.);
#12459=FACE_OUTER_BOUND('',#18619,.T.);
#12460=FACE_OUTER_BOUND('',#18620,.T.);
#12461=FACE_OUTER_BOUND('',#18621,.T.);
#12462=FACE_OUTER_BOUND('',#18622,.T.);
#12463=FACE_OUTER_BOUND('',#18623,.T.);
#12464=FACE_OUTER_BOUND('',#18624,.T.);
#12465=FACE_OUTER_BOUND('',#18625,.T.);
#12466=FACE_OUTER_BOUND('',#18626,.T.);
#12467=FACE_OUTER_BOUND('',#18627,.T.);
#12468=FACE_OUTER_BOUND('',#18628,.T.);
#12469=FACE_OUTER_BOUND('',#18629,.T.);
#12470=FACE_OUTER_BOUND('',#18630,.T.);
#12471=FACE_OUTER_BOUND('',#18631,.T.);
#12472=FACE_OUTER_BOUND('',#18632,.T.);
#12473=FACE_OUTER_BOUND('',#18633,.T.);
#12474=FACE_OUTER_BOUND('',#18634,.T.);
#12475=FACE_OUTER_BOUND('',#18635,.T.);
#12476=FACE_OUTER_BOUND('',#18636,.T.);
#12477=FACE_OUTER_BOUND('',#18637,.T.);
#12478=FACE_OUTER_BOUND('',#18638,.T.);
#12479=FACE_OUTER_BOUND('',#18639,.T.);
#12480=FACE_OUTER_BOUND('',#18640,.T.);
#12481=FACE_OUTER_BOUND('',#18641,.T.);
#12482=FACE_OUTER_BOUND('',#18642,.T.);
#12483=FACE_OUTER_BOUND('',#18643,.T.);
#12484=FACE_OUTER_BOUND('',#18644,.T.);
#12485=FACE_OUTER_BOUND('',#18645,.T.);
#12486=FACE_OUTER_BOUND('',#18646,.T.);
#12487=FACE_OUTER_BOUND('',#18647,.T.);
#12488=FACE_OUTER_BOUND('',#18648,.T.);
#12489=FACE_OUTER_BOUND('',#18649,.T.);
#12490=FACE_OUTER_BOUND('',#18650,.T.);
#12491=FACE_OUTER_BOUND('',#18651,.T.);
#12492=FACE_OUTER_BOUND('',#18652,.T.);
#12493=FACE_OUTER_BOUND('',#18653,.T.);
#12494=FACE_OUTER_BOUND('',#18654,.T.);
#12495=FACE_OUTER_BOUND('',#18655,.T.);
#12496=FACE_OUTER_BOUND('',#18656,.T.);
#12497=FACE_OUTER_BOUND('',#18657,.T.);
#12498=FACE_OUTER_BOUND('',#18658,.T.);
#12499=FACE_OUTER_BOUND('',#18659,.T.);
#12500=FACE_OUTER_BOUND('',#18660,.T.);
#12501=FACE_OUTER_BOUND('',#18661,.T.);
#12502=FACE_OUTER_BOUND('',#18662,.T.);
#12503=FACE_OUTER_BOUND('',#18663,.T.);
#12504=FACE_OUTER_BOUND('',#18664,.T.);
#12505=FACE_OUTER_BOUND('',#18665,.T.);
#12506=FACE_OUTER_BOUND('',#18666,.T.);
#12507=FACE_OUTER_BOUND('',#18667,.T.);
#12508=FACE_OUTER_BOUND('',#18668,.T.);
#12509=FACE_OUTER_BOUND('',#18669,.T.);
#12510=FACE_OUTER_BOUND('',#18670,.T.);
#12511=FACE_OUTER_BOUND('',#18671,.T.);
#12512=FACE_OUTER_BOUND('',#18672,.T.);
#12513=FACE_OUTER_BOUND('',#18673,.T.);
#12514=FACE_OUTER_BOUND('',#18674,.T.);
#12515=FACE_OUTER_BOUND('',#18675,.T.);
#12516=FACE_OUTER_BOUND('',#18676,.T.);
#12517=FACE_OUTER_BOUND('',#18677,.T.);
#12518=FACE_OUTER_BOUND('',#18678,.T.);
#12519=FACE_OUTER_BOUND('',#18679,.T.);
#12520=FACE_OUTER_BOUND('',#18680,.T.);
#12521=FACE_OUTER_BOUND('',#18681,.T.);
#12522=FACE_OUTER_BOUND('',#18682,.T.);
#12523=FACE_OUTER_BOUND('',#18683,.T.);
#12524=FACE_OUTER_BOUND('',#18684,.T.);
#12525=FACE_OUTER_BOUND('',#18685,.T.);
#12526=FACE_OUTER_BOUND('',#18686,.T.);
#12527=FACE_OUTER_BOUND('',#18687,.T.);
#12528=FACE_OUTER_BOUND('',#18688,.T.);
#12529=FACE_OUTER_BOUND('',#18689,.T.);
#12530=FACE_OUTER_BOUND('',#18690,.T.);
#12531=FACE_OUTER_BOUND('',#18691,.T.);
#12532=FACE_OUTER_BOUND('',#18692,.T.);
#12533=FACE_OUTER_BOUND('',#18693,.T.);
#12534=FACE_OUTER_BOUND('',#18694,.T.);
#12535=FACE_OUTER_BOUND('',#18695,.T.);
#12536=FACE_OUTER_BOUND('',#18696,.T.);
#12537=FACE_OUTER_BOUND('',#18697,.T.);
#12538=FACE_OUTER_BOUND('',#18698,.T.);
#12539=FACE_OUTER_BOUND('',#18699,.T.);
#12540=FACE_OUTER_BOUND('',#18700,.T.);
#12541=FACE_OUTER_BOUND('',#18701,.T.);
#12542=FACE_OUTER_BOUND('',#18702,.T.);
#12543=FACE_OUTER_BOUND('',#18703,.T.);
#12544=FACE_OUTER_BOUND('',#18704,.T.);
#12545=FACE_OUTER_BOUND('',#18705,.T.);
#12546=FACE_OUTER_BOUND('',#18706,.T.);
#12547=FACE_OUTER_BOUND('',#18707,.T.);
#12548=FACE_OUTER_BOUND('',#18708,.T.);
#12549=FACE_OUTER_BOUND('',#18709,.T.);
#12550=FACE_OUTER_BOUND('',#18710,.T.);
#12551=FACE_OUTER_BOUND('',#18711,.T.);
#12552=FACE_OUTER_BOUND('',#18712,.T.);
#12553=FACE_OUTER_BOUND('',#18713,.T.);
#12554=FACE_OUTER_BOUND('',#18714,.T.);
#12555=FACE_OUTER_BOUND('',#18715,.T.);
#12556=FACE_OUTER_BOUND('',#18716,.T.);
#12557=FACE_OUTER_BOUND('',#18717,.T.);
#12558=FACE_OUTER_BOUND('',#18718,.T.);
#12559=FACE_OUTER_BOUND('',#18719,.T.);
#12560=FACE_OUTER_BOUND('',#18720,.T.);
#12561=FACE_OUTER_BOUND('',#18721,.T.);
#12562=FACE_OUTER_BOUND('',#18722,.T.);
#12563=FACE_OUTER_BOUND('',#18723,.T.);
#12564=FACE_OUTER_BOUND('',#18724,.T.);
#12565=FACE_OUTER_BOUND('',#18725,.T.);
#12566=FACE_OUTER_BOUND('',#18726,.T.);
#12567=FACE_OUTER_BOUND('',#18727,.T.);
#12568=FACE_OUTER_BOUND('',#18728,.T.);
#12569=FACE_OUTER_BOUND('',#18729,.T.);
#12570=FACE_OUTER_BOUND('',#18730,.T.);
#12571=FACE_OUTER_BOUND('',#18731,.T.);
#12572=FACE_OUTER_BOUND('',#18732,.T.);
#12573=FACE_OUTER_BOUND('',#18733,.T.);
#12574=FACE_OUTER_BOUND('',#18734,.T.);
#12575=FACE_OUTER_BOUND('',#18735,.T.);
#12576=FACE_OUTER_BOUND('',#18736,.T.);
#12577=FACE_OUTER_BOUND('',#18737,.T.);
#12578=FACE_OUTER_BOUND('',#18738,.T.);
#12579=FACE_OUTER_BOUND('',#18739,.T.);
#12580=FACE_OUTER_BOUND('',#18740,.T.);
#12581=FACE_OUTER_BOUND('',#18741,.T.);
#12582=FACE_OUTER_BOUND('',#18742,.T.);
#12583=FACE_OUTER_BOUND('',#18743,.T.);
#12584=FACE_OUTER_BOUND('',#18744,.T.);
#12585=FACE_OUTER_BOUND('',#18745,.T.);
#12586=FACE_OUTER_BOUND('',#18746,.T.);
#12587=FACE_OUTER_BOUND('',#18747,.T.);
#12588=FACE_OUTER_BOUND('',#18748,.T.);
#12589=FACE_OUTER_BOUND('',#18749,.T.);
#12590=FACE_OUTER_BOUND('',#18750,.T.);
#12591=FACE_OUTER_BOUND('',#18751,.T.);
#12592=FACE_OUTER_BOUND('',#18752,.T.);
#12593=FACE_OUTER_BOUND('',#18753,.T.);
#12594=FACE_OUTER_BOUND('',#18754,.T.);
#12595=FACE_OUTER_BOUND('',#18755,.T.);
#12596=FACE_OUTER_BOUND('',#18756,.T.);
#12597=FACE_OUTER_BOUND('',#18757,.T.);
#12598=FACE_OUTER_BOUND('',#18758,.T.);
#12599=FACE_OUTER_BOUND('',#18759,.T.);
#12600=FACE_OUTER_BOUND('',#18760,.T.);
#12601=FACE_OUTER_BOUND('',#18761,.T.);
#12602=FACE_OUTER_BOUND('',#18762,.T.);
#12603=FACE_OUTER_BOUND('',#18763,.T.);
#12604=FACE_OUTER_BOUND('',#18764,.T.);
#12605=FACE_OUTER_BOUND('',#18765,.T.);
#12606=FACE_OUTER_BOUND('',#18766,.T.);
#12607=FACE_OUTER_BOUND('',#18767,.T.);
#12608=FACE_OUTER_BOUND('',#18768,.T.);
#12609=FACE_OUTER_BOUND('',#18769,.T.);
#12610=FACE_OUTER_BOUND('',#18770,.T.);
#12611=FACE_OUTER_BOUND('',#18771,.T.);
#12612=FACE_OUTER_BOUND('',#18772,.T.);
#12613=FACE_OUTER_BOUND('',#18773,.T.);
#12614=FACE_OUTER_BOUND('',#18774,.T.);
#12615=FACE_OUTER_BOUND('',#18775,.T.);
#12616=FACE_OUTER_BOUND('',#18776,.T.);
#12617=FACE_OUTER_BOUND('',#18777,.T.);
#12618=FACE_OUTER_BOUND('',#18778,.T.);
#12619=FACE_OUTER_BOUND('',#18779,.T.);
#12620=FACE_OUTER_BOUND('',#18780,.T.);
#12621=FACE_OUTER_BOUND('',#18781,.T.);
#12622=FACE_OUTER_BOUND('',#18782,.T.);
#12623=FACE_OUTER_BOUND('',#18783,.T.);
#12624=FACE_OUTER_BOUND('',#18784,.T.);
#12625=FACE_OUTER_BOUND('',#18785,.T.);
#12626=FACE_OUTER_BOUND('',#18786,.T.);
#12627=FACE_OUTER_BOUND('',#18787,.T.);
#12628=FACE_OUTER_BOUND('',#18788,.T.);
#12629=FACE_OUTER_BOUND('',#18789,.T.);
#12630=FACE_OUTER_BOUND('',#18790,.T.);
#12631=FACE_OUTER_BOUND('',#18791,.T.);
#12632=FACE_OUTER_BOUND('',#18792,.T.);
#12633=FACE_OUTER_BOUND('',#18793,.T.);
#12634=FACE_OUTER_BOUND('',#18794,.T.);
#12635=FACE_OUTER_BOUND('',#18795,.T.);
#12636=FACE_OUTER_BOUND('',#18796,.T.);
#12637=FACE_OUTER_BOUND('',#18797,.T.);
#12638=FACE_OUTER_BOUND('',#18798,.T.);
#12639=FACE_OUTER_BOUND('',#18799,.T.);
#12640=FACE_OUTER_BOUND('',#18800,.T.);
#12641=FACE_OUTER_BOUND('',#18801,.T.);
#12642=FACE_OUTER_BOUND('',#18802,.T.);
#12643=FACE_OUTER_BOUND('',#18803,.T.);
#12644=FACE_OUTER_BOUND('',#18804,.T.);
#12645=FACE_OUTER_BOUND('',#18805,.T.);
#12646=FACE_OUTER_BOUND('',#18806,.T.);
#12647=FACE_OUTER_BOUND('',#18807,.T.);
#12648=FACE_OUTER_BOUND('',#18808,.T.);
#12649=FACE_OUTER_BOUND('',#18809,.T.);
#12650=FACE_OUTER_BOUND('',#18810,.T.);
#12651=FACE_OUTER_BOUND('',#18811,.T.);
#12652=FACE_OUTER_BOUND('',#18812,.T.);
#12653=FACE_OUTER_BOUND('',#18813,.T.);
#12654=FACE_OUTER_BOUND('',#18814,.T.);
#12655=FACE_OUTER_BOUND('',#18815,.T.);
#12656=FACE_OUTER_BOUND('',#18816,.T.);
#12657=FACE_OUTER_BOUND('',#18817,.T.);
#12658=FACE_OUTER_BOUND('',#18818,.T.);
#12659=FACE_OUTER_BOUND('',#18819,.T.);
#12660=FACE_OUTER_BOUND('',#18820,.T.);
#12661=FACE_OUTER_BOUND('',#18821,.T.);
#12662=FACE_OUTER_BOUND('',#18822,.T.);
#12663=FACE_OUTER_BOUND('',#18823,.T.);
#12664=FACE_OUTER_BOUND('',#18824,.T.);
#12665=FACE_OUTER_BOUND('',#18825,.T.);
#12666=FACE_OUTER_BOUND('',#18826,.T.);
#12667=FACE_OUTER_BOUND('',#18827,.T.);
#12668=FACE_OUTER_BOUND('',#18828,.T.);
#12669=FACE_OUTER_BOUND('',#18829,.T.);
#12670=FACE_OUTER_BOUND('',#18830,.T.);
#12671=FACE_OUTER_BOUND('',#18831,.T.);
#12672=FACE_OUTER_BOUND('',#18832,.T.);
#12673=FACE_OUTER_BOUND('',#18833,.T.);
#12674=FACE_OUTER_BOUND('',#18834,.T.);
#12675=FACE_OUTER_BOUND('',#18835,.T.);
#12676=FACE_OUTER_BOUND('',#18836,.T.);
#12677=FACE_OUTER_BOUND('',#18837,.T.);
#12678=FACE_OUTER_BOUND('',#18838,.T.);
#12679=FACE_OUTER_BOUND('',#18839,.T.);
#12680=FACE_OUTER_BOUND('',#18840,.T.);
#12681=FACE_OUTER_BOUND('',#18841,.T.);
#12682=FACE_OUTER_BOUND('',#18842,.T.);
#12683=FACE_OUTER_BOUND('',#18843,.T.);
#12684=FACE_OUTER_BOUND('',#18844,.T.);
#12685=FACE_OUTER_BOUND('',#18845,.T.);
#12686=FACE_OUTER_BOUND('',#18846,.T.);
#12687=FACE_OUTER_BOUND('',#18847,.T.);
#12688=FACE_OUTER_BOUND('',#18848,.T.);
#12689=FACE_OUTER_BOUND('',#18849,.T.);
#12690=FACE_OUTER_BOUND('',#18850,.T.);
#12691=FACE_OUTER_BOUND('',#18851,.T.);
#12692=FACE_OUTER_BOUND('',#18852,.T.);
#12693=FACE_OUTER_BOUND('',#18853,.T.);
#12694=FACE_OUTER_BOUND('',#18854,.T.);
#12695=FACE_OUTER_BOUND('',#18855,.T.);
#12696=FACE_OUTER_BOUND('',#18856,.T.);
#12697=FACE_OUTER_BOUND('',#18857,.T.);
#12698=FACE_OUTER_BOUND('',#18858,.T.);
#12699=FACE_OUTER_BOUND('',#18859,.T.);
#12700=FACE_OUTER_BOUND('',#18860,.T.);
#12701=FACE_OUTER_BOUND('',#18861,.T.);
#12702=FACE_OUTER_BOUND('',#18862,.T.);
#12703=FACE_OUTER_BOUND('',#18863,.T.);
#12704=FACE_OUTER_BOUND('',#18864,.T.);
#12705=FACE_OUTER_BOUND('',#18865,.T.);
#12706=FACE_OUTER_BOUND('',#18866,.T.);
#12707=FACE_OUTER_BOUND('',#18867,.T.);
#12708=FACE_OUTER_BOUND('',#18868,.T.);
#12709=FACE_OUTER_BOUND('',#18869,.T.);
#12710=FACE_OUTER_BOUND('',#18870,.T.);
#12711=FACE_OUTER_BOUND('',#18871,.T.);
#12712=FACE_OUTER_BOUND('',#18872,.T.);
#12713=FACE_OUTER_BOUND('',#18873,.T.);
#12714=FACE_OUTER_BOUND('',#18874,.T.);
#12715=FACE_OUTER_BOUND('',#18875,.T.);
#12716=FACE_OUTER_BOUND('',#18876,.T.);
#12717=FACE_OUTER_BOUND('',#18877,.T.);
#12718=FACE_OUTER_BOUND('',#18878,.T.);
#12719=FACE_OUTER_BOUND('',#18879,.T.);
#12720=FACE_OUTER_BOUND('',#18880,.T.);
#12721=FACE_OUTER_BOUND('',#18881,.T.);
#12722=FACE_OUTER_BOUND('',#18882,.T.);
#12723=FACE_OUTER_BOUND('',#18883,.T.);
#12724=FACE_OUTER_BOUND('',#18884,.T.);
#12725=FACE_OUTER_BOUND('',#18885,.T.);
#12726=FACE_OUTER_BOUND('',#18886,.T.);
#12727=FACE_OUTER_BOUND('',#18887,.T.);
#12728=FACE_OUTER_BOUND('',#18888,.T.);
#12729=FACE_OUTER_BOUND('',#18889,.T.);
#12730=FACE_OUTER_BOUND('',#18890,.T.);
#12731=FACE_OUTER_BOUND('',#18891,.T.);
#12732=FACE_OUTER_BOUND('',#18892,.T.);
#12733=FACE_OUTER_BOUND('',#18893,.T.);
#12734=FACE_OUTER_BOUND('',#18894,.T.);
#12735=FACE_OUTER_BOUND('',#18895,.T.);
#12736=FACE_OUTER_BOUND('',#18896,.T.);
#12737=FACE_OUTER_BOUND('',#18897,.T.);
#12738=FACE_OUTER_BOUND('',#18898,.T.);
#12739=FACE_OUTER_BOUND('',#18899,.T.);
#12740=FACE_OUTER_BOUND('',#18900,.T.);
#12741=FACE_OUTER_BOUND('',#18901,.T.);
#12742=FACE_OUTER_BOUND('',#18902,.T.);
#12743=FACE_OUTER_BOUND('',#18903,.T.);
#12744=FACE_OUTER_BOUND('',#18904,.T.);
#12745=FACE_OUTER_BOUND('',#18905,.T.);
#12746=FACE_OUTER_BOUND('',#18906,.T.);
#12747=FACE_OUTER_BOUND('',#18907,.T.);
#12748=FACE_OUTER_BOUND('',#18908,.T.);
#12749=FACE_OUTER_BOUND('',#18909,.T.);
#12750=FACE_OUTER_BOUND('',#18910,.T.);
#12751=FACE_OUTER_BOUND('',#18911,.T.);
#12752=FACE_OUTER_BOUND('',#18912,.T.);
#12753=FACE_OUTER_BOUND('',#18913,.T.);
#12754=FACE_OUTER_BOUND('',#18914,.T.);
#12755=FACE_OUTER_BOUND('',#18915,.T.);
#12756=FACE_OUTER_BOUND('',#18916,.T.);
#12757=FACE_OUTER_BOUND('',#18917,.T.);
#12758=FACE_OUTER_BOUND('',#18918,.T.);
#12759=FACE_OUTER_BOUND('',#18919,.T.);
#12760=FACE_OUTER_BOUND('',#18920,.T.);
#12761=FACE_OUTER_BOUND('',#18921,.T.);
#12762=FACE_OUTER_BOUND('',#18922,.T.);
#12763=FACE_OUTER_BOUND('',#18923,.T.);
#12764=FACE_OUTER_BOUND('',#18924,.T.);
#12765=FACE_OUTER_BOUND('',#18925,.T.);
#12766=FACE_OUTER_BOUND('',#18926,.T.);
#12767=FACE_OUTER_BOUND('',#18927,.T.);
#12768=FACE_OUTER_BOUND('',#18928,.T.);
#12769=FACE_OUTER_BOUND('',#18929,.T.);
#12770=FACE_OUTER_BOUND('',#18930,.T.);
#12771=FACE_OUTER_BOUND('',#18931,.T.);
#12772=FACE_OUTER_BOUND('',#18932,.T.);
#12773=FACE_OUTER_BOUND('',#18933,.T.);
#12774=FACE_OUTER_BOUND('',#18934,.T.);
#12775=FACE_OUTER_BOUND('',#18935,.T.);
#12776=FACE_OUTER_BOUND('',#18936,.T.);
#12777=FACE_OUTER_BOUND('',#18937,.T.);
#12778=FACE_OUTER_BOUND('',#18938,.T.);
#12779=FACE_OUTER_BOUND('',#18939,.T.);
#12780=FACE_OUTER_BOUND('',#18940,.T.);
#12781=FACE_OUTER_BOUND('',#18941,.T.);
#12782=FACE_OUTER_BOUND('',#18942,.T.);
#12783=FACE_OUTER_BOUND('',#18943,.T.);
#12784=FACE_OUTER_BOUND('',#18944,.T.);
#12785=FACE_OUTER_BOUND('',#18945,.T.);
#12786=FACE_OUTER_BOUND('',#18946,.T.);
#12787=FACE_OUTER_BOUND('',#18947,.T.);
#12788=FACE_OUTER_BOUND('',#18948,.T.);
#12789=FACE_OUTER_BOUND('',#18949,.T.);
#12790=FACE_OUTER_BOUND('',#18950,.T.);
#12791=FACE_OUTER_BOUND('',#18951,.T.);
#12792=FACE_OUTER_BOUND('',#18952,.T.);
#12793=FACE_OUTER_BOUND('',#18953,.T.);
#12794=FACE_OUTER_BOUND('',#18954,.T.);
#12795=FACE_OUTER_BOUND('',#18955,.T.);
#12796=FACE_OUTER_BOUND('',#18956,.T.);
#12797=FACE_OUTER_BOUND('',#18957,.T.);
#12798=FACE_OUTER_BOUND('',#18958,.T.);
#12799=FACE_OUTER_BOUND('',#18959,.T.);
#12800=FACE_OUTER_BOUND('',#18960,.T.);
#12801=FACE_OUTER_BOUND('',#18961,.T.);
#12802=FACE_OUTER_BOUND('',#18962,.T.);
#12803=FACE_OUTER_BOUND('',#18963,.T.);
#12804=FACE_OUTER_BOUND('',#18964,.T.);
#12805=FACE_OUTER_BOUND('',#18965,.T.);
#12806=FACE_OUTER_BOUND('',#18966,.T.);
#12807=FACE_OUTER_BOUND('',#18967,.T.);
#12808=FACE_OUTER_BOUND('',#18968,.T.);
#12809=FACE_OUTER_BOUND('',#18969,.T.);
#12810=FACE_OUTER_BOUND('',#18970,.T.);
#12811=FACE_OUTER_BOUND('',#18971,.T.);
#12812=FACE_OUTER_BOUND('',#18972,.T.);
#12813=FACE_OUTER_BOUND('',#18973,.T.);
#12814=FACE_OUTER_BOUND('',#18974,.T.);
#12815=FACE_OUTER_BOUND('',#18975,.T.);
#12816=FACE_OUTER_BOUND('',#18976,.T.);
#12817=FACE_OUTER_BOUND('',#18977,.T.);
#12818=FACE_OUTER_BOUND('',#18978,.T.);
#12819=FACE_OUTER_BOUND('',#18979,.T.);
#12820=FACE_OUTER_BOUND('',#18980,.T.);
#12821=FACE_OUTER_BOUND('',#18981,.T.);
#12822=FACE_OUTER_BOUND('',#18982,.T.);
#12823=FACE_OUTER_BOUND('',#18983,.T.);
#12824=FACE_OUTER_BOUND('',#18984,.T.);
#12825=FACE_OUTER_BOUND('',#18985,.T.);
#12826=FACE_OUTER_BOUND('',#18986,.T.);
#12827=FACE_OUTER_BOUND('',#18987,.T.);
#12828=FACE_OUTER_BOUND('',#18988,.T.);
#12829=FACE_OUTER_BOUND('',#18989,.T.);
#12830=FACE_OUTER_BOUND('',#18990,.T.);
#12831=FACE_OUTER_BOUND('',#18991,.T.);
#12832=FACE_OUTER_BOUND('',#18992,.T.);
#12833=FACE_OUTER_BOUND('',#18993,.T.);
#12834=FACE_OUTER_BOUND('',#18994,.T.);
#12835=FACE_OUTER_BOUND('',#18995,.T.);
#12836=FACE_OUTER_BOUND('',#18996,.T.);
#12837=FACE_OUTER_BOUND('',#18997,.T.);
#12838=FACE_OUTER_BOUND('',#18998,.T.);
#12839=FACE_OUTER_BOUND('',#18999,.T.);
#12840=FACE_OUTER_BOUND('',#19000,.T.);
#12841=FACE_OUTER_BOUND('',#19001,.T.);
#12842=FACE_OUTER_BOUND('',#19002,.T.);
#12843=FACE_OUTER_BOUND('',#19003,.T.);
#12844=FACE_OUTER_BOUND('',#19004,.T.);
#12845=FACE_OUTER_BOUND('',#19005,.T.);
#12846=FACE_OUTER_BOUND('',#19006,.T.);
#12847=FACE_OUTER_BOUND('',#19007,.T.);
#12848=FACE_OUTER_BOUND('',#19009,.T.);
#12849=FACE_OUTER_BOUND('',#19011,.T.);
#12850=FACE_OUTER_BOUND('',#19013,.T.);
#12851=FACE_OUTER_BOUND('',#19014,.T.);
#12852=FACE_OUTER_BOUND('',#19015,.T.);
#12853=FACE_OUTER_BOUND('',#19016,.T.);
#12854=FACE_OUTER_BOUND('',#19017,.T.);
#12855=FACE_OUTER_BOUND('',#19019,.T.);
#12856=FACE_OUTER_BOUND('',#19021,.T.);
#12857=FACE_OUTER_BOUND('',#19022,.T.);
#12858=FACE_OUTER_BOUND('',#19023,.T.);
#12859=FACE_OUTER_BOUND('',#19024,.T.);
#12860=FACE_OUTER_BOUND('',#19025,.T.);
#12861=FACE_OUTER_BOUND('',#19026,.T.);
#12862=FACE_OUTER_BOUND('',#19027,.T.);
#12863=FACE_OUTER_BOUND('',#19028,.T.);
#12864=FACE_OUTER_BOUND('',#19029,.T.);
#12865=FACE_OUTER_BOUND('',#19030,.T.);
#12866=FACE_OUTER_BOUND('',#19031,.T.);
#12867=FACE_OUTER_BOUND('',#19032,.T.);
#12868=FACE_OUTER_BOUND('',#19033,.T.);
#12869=FACE_OUTER_BOUND('',#19034,.T.);
#12870=FACE_OUTER_BOUND('',#19035,.T.);
#12871=FACE_OUTER_BOUND('',#19036,.T.);
#12872=FACE_OUTER_BOUND('',#19037,.T.);
#12873=FACE_OUTER_BOUND('',#19038,.T.);
#12874=FACE_OUTER_BOUND('',#19039,.T.);
#12875=FACE_OUTER_BOUND('',#19040,.T.);
#12876=FACE_OUTER_BOUND('',#19041,.T.);
#12877=FACE_OUTER_BOUND('',#19042,.T.);
#12878=FACE_OUTER_BOUND('',#19043,.T.);
#12879=FACE_OUTER_BOUND('',#19044,.T.);
#12880=FACE_OUTER_BOUND('',#19045,.T.);
#12881=FACE_OUTER_BOUND('',#19046,.T.);
#12882=FACE_OUTER_BOUND('',#19047,.T.);
#12883=FACE_OUTER_BOUND('',#19048,.T.);
#12884=FACE_OUTER_BOUND('',#19049,.T.);
#12885=FACE_OUTER_BOUND('',#19050,.T.);
#12886=FACE_OUTER_BOUND('',#19051,.T.);
#12887=FACE_OUTER_BOUND('',#19052,.T.);
#12888=FACE_OUTER_BOUND('',#19053,.T.);
#12889=FACE_OUTER_BOUND('',#19054,.T.);
#12890=FACE_OUTER_BOUND('',#19055,.T.);
#12891=FACE_OUTER_BOUND('',#19056,.T.);
#12892=FACE_OUTER_BOUND('',#19058,.T.);
#12893=FACE_OUTER_BOUND('',#19059,.T.);
#12894=FACE_OUTER_BOUND('',#19060,.T.);
#12895=FACE_OUTER_BOUND('',#19061,.T.);
#12896=FACE_OUTER_BOUND('',#19062,.T.);
#12897=FACE_OUTER_BOUND('',#19063,.T.);
#12898=FACE_OUTER_BOUND('',#19064,.T.);
#12899=FACE_OUTER_BOUND('',#19065,.T.);
#12900=FACE_OUTER_BOUND('',#19066,.T.);
#12901=FACE_OUTER_BOUND('',#19068,.T.);
#12902=FACE_OUTER_BOUND('',#19069,.T.);
#12903=FACE_OUTER_BOUND('',#19071,.T.);
#12904=FACE_OUTER_BOUND('',#19072,.T.);
#12905=FACE_OUTER_BOUND('',#19074,.T.);
#12906=FACE_OUTER_BOUND('',#19076,.T.);
#12907=FACE_OUTER_BOUND('',#19077,.T.);
#12908=FACE_OUTER_BOUND('',#19078,.T.);
#12909=FACE_OUTER_BOUND('',#19079,.T.);
#12910=FACE_OUTER_BOUND('',#19080,.T.);
#12911=FACE_OUTER_BOUND('',#19081,.T.);
#12912=FACE_OUTER_BOUND('',#19082,.T.);
#12913=FACE_OUTER_BOUND('',#19083,.T.);
#12914=FACE_OUTER_BOUND('',#19084,.T.);
#12915=FACE_OUTER_BOUND('',#19085,.T.);
#12916=FACE_OUTER_BOUND('',#19086,.T.);
#12917=FACE_OUTER_BOUND('',#19087,.T.);
#12918=FACE_OUTER_BOUND('',#19093,.T.);
#12919=FACE_OUTER_BOUND('',#19095,.T.);
#12920=FACE_OUTER_BOUND('',#19097,.T.);
#12921=FACE_OUTER_BOUND('',#19098,.T.);
#12922=FACE_OUTER_BOUND('',#19099,.T.);
#12923=FACE_OUTER_BOUND('',#19100,.T.);
#12924=FACE_OUTER_BOUND('',#19101,.T.);
#12925=FACE_OUTER_BOUND('',#19102,.T.);
#12926=FACE_OUTER_BOUND('',#19103,.T.);
#12927=FACE_OUTER_BOUND('',#19104,.T.);
#12928=FACE_OUTER_BOUND('',#19105,.T.);
#12929=FACE_OUTER_BOUND('',#19106,.T.);
#12930=FACE_OUTER_BOUND('',#19107,.T.);
#12931=FACE_OUTER_BOUND('',#19108,.T.);
#12932=FACE_OUTER_BOUND('',#19109,.T.);
#12933=FACE_OUTER_BOUND('',#19110,.T.);
#12934=FACE_OUTER_BOUND('',#19111,.T.);
#12935=FACE_OUTER_BOUND('',#19112,.T.);
#12936=FACE_OUTER_BOUND('',#19113,.T.);
#12937=FACE_OUTER_BOUND('',#19114,.T.);
#12938=FACE_OUTER_BOUND('',#19115,.T.);
#12939=FACE_OUTER_BOUND('',#19116,.T.);
#12940=FACE_OUTER_BOUND('',#19117,.T.);
#12941=FACE_OUTER_BOUND('',#19118,.T.);
#12942=FACE_OUTER_BOUND('',#19119,.T.);
#12943=FACE_OUTER_BOUND('',#19120,.T.);
#12944=FACE_OUTER_BOUND('',#19121,.T.);
#12945=FACE_OUTER_BOUND('',#19122,.T.);
#12946=FACE_OUTER_BOUND('',#19123,.T.);
#12947=FACE_OUTER_BOUND('',#19124,.T.);
#12948=FACE_OUTER_BOUND('',#19125,.T.);
#12949=FACE_OUTER_BOUND('',#19126,.T.);
#12950=FACE_OUTER_BOUND('',#19127,.T.);
#12951=FACE_OUTER_BOUND('',#19128,.T.);
#12952=FACE_OUTER_BOUND('',#19129,.T.);
#12953=FACE_OUTER_BOUND('',#19130,.T.);
#12954=FACE_OUTER_BOUND('',#19131,.T.);
#12955=FACE_OUTER_BOUND('',#19132,.T.);
#12956=FACE_OUTER_BOUND('',#19133,.T.);
#12957=FACE_OUTER_BOUND('',#19134,.T.);
#12958=FACE_OUTER_BOUND('',#19135,.T.);
#12959=FACE_OUTER_BOUND('',#19136,.T.);
#12960=FACE_OUTER_BOUND('',#19137,.T.);
#12961=FACE_OUTER_BOUND('',#19138,.T.);
#12962=FACE_OUTER_BOUND('',#19139,.T.);
#12963=FACE_OUTER_BOUND('',#19140,.T.);
#12964=FACE_OUTER_BOUND('',#19141,.T.);
#12965=FACE_OUTER_BOUND('',#19142,.T.);
#12966=FACE_OUTER_BOUND('',#19143,.T.);
#12967=FACE_OUTER_BOUND('',#19144,.T.);
#12968=FACE_OUTER_BOUND('',#19145,.T.);
#12969=FACE_OUTER_BOUND('',#19146,.T.);
#12970=FACE_OUTER_BOUND('',#19147,.T.);
#12971=FACE_OUTER_BOUND('',#19148,.T.);
#12972=FACE_OUTER_BOUND('',#19149,.T.);
#12973=FACE_OUTER_BOUND('',#19150,.T.);
#12974=FACE_OUTER_BOUND('',#19151,.T.);
#12975=FACE_OUTER_BOUND('',#19152,.T.);
#12976=FACE_OUTER_BOUND('',#19153,.T.);
#12977=FACE_OUTER_BOUND('',#19154,.T.);
#12978=FACE_OUTER_BOUND('',#19155,.T.);
#12979=FACE_OUTER_BOUND('',#19156,.T.);
#12980=FACE_OUTER_BOUND('',#19157,.T.);
#12981=FACE_OUTER_BOUND('',#19158,.T.);
#12982=FACE_OUTER_BOUND('',#19159,.T.);
#12983=FACE_OUTER_BOUND('',#19160,.T.);
#12984=FACE_OUTER_BOUND('',#19161,.T.);
#12985=FACE_OUTER_BOUND('',#19162,.T.);
#12986=FACE_OUTER_BOUND('',#19163,.T.);
#12987=FACE_OUTER_BOUND('',#19164,.T.);
#12988=FACE_OUTER_BOUND('',#19165,.T.);
#12989=FACE_OUTER_BOUND('',#19166,.T.);
#12990=FACE_OUTER_BOUND('',#19167,.T.);
#12991=FACE_OUTER_BOUND('',#19168,.T.);
#12992=FACE_OUTER_BOUND('',#19169,.T.);
#12993=FACE_OUTER_BOUND('',#19170,.T.);
#12994=FACE_OUTER_BOUND('',#19171,.T.);
#12995=FACE_OUTER_BOUND('',#19172,.T.);
#12996=FACE_OUTER_BOUND('',#19173,.T.);
#12997=FACE_OUTER_BOUND('',#19174,.T.);
#12998=FACE_OUTER_BOUND('',#19175,.T.);
#12999=FACE_OUTER_BOUND('',#19176,.T.);
#13000=FACE_OUTER_BOUND('',#19177,.T.);
#13001=FACE_OUTER_BOUND('',#19178,.T.);
#13002=FACE_OUTER_BOUND('',#19179,.T.);
#13003=FACE_OUTER_BOUND('',#19180,.T.);
#13004=FACE_OUTER_BOUND('',#19181,.T.);
#13005=FACE_OUTER_BOUND('',#19182,.T.);
#13006=FACE_OUTER_BOUND('',#19183,.T.);
#13007=FACE_OUTER_BOUND('',#19184,.T.);
#13008=FACE_OUTER_BOUND('',#19185,.T.);
#13009=FACE_OUTER_BOUND('',#19186,.T.);
#13010=FACE_OUTER_BOUND('',#19187,.T.);
#13011=FACE_OUTER_BOUND('',#19188,.T.);
#13012=FACE_OUTER_BOUND('',#19189,.T.);
#13013=FACE_OUTER_BOUND('',#19190,.T.);
#13014=FACE_OUTER_BOUND('',#19191,.T.);
#13015=FACE_OUTER_BOUND('',#19192,.T.);
#13016=FACE_OUTER_BOUND('',#19193,.T.);
#13017=FACE_OUTER_BOUND('',#19194,.T.);
#13018=FACE_OUTER_BOUND('',#19195,.T.);
#13019=FACE_OUTER_BOUND('',#19196,.T.);
#13020=FACE_OUTER_BOUND('',#19197,.T.);
#13021=FACE_OUTER_BOUND('',#19198,.T.);
#13022=FACE_OUTER_BOUND('',#19199,.T.);
#13023=FACE_OUTER_BOUND('',#19200,.T.);
#13024=FACE_OUTER_BOUND('',#19201,.T.);
#13025=FACE_OUTER_BOUND('',#19202,.T.);
#13026=FACE_OUTER_BOUND('',#19203,.T.);
#13027=FACE_OUTER_BOUND('',#19204,.T.);
#13028=FACE_OUTER_BOUND('',#19205,.T.);
#13029=FACE_OUTER_BOUND('',#19206,.T.);
#13030=FACE_OUTER_BOUND('',#19207,.T.);
#13031=FACE_OUTER_BOUND('',#19208,.T.);
#13032=FACE_OUTER_BOUND('',#19209,.T.);
#13033=FACE_OUTER_BOUND('',#19210,.T.);
#13034=FACE_OUTER_BOUND('',#19211,.T.);
#13035=FACE_OUTER_BOUND('',#19212,.T.);
#13036=FACE_OUTER_BOUND('',#19213,.T.);
#13037=FACE_OUTER_BOUND('',#19214,.T.);
#13038=FACE_OUTER_BOUND('',#19215,.T.);
#13039=FACE_OUTER_BOUND('',#19217,.T.);
#13040=FACE_OUTER_BOUND('',#19218,.T.);
#13041=FACE_OUTER_BOUND('',#19219,.T.);
#13042=FACE_OUTER_BOUND('',#19220,.T.);
#13043=FACE_OUTER_BOUND('',#19221,.T.);
#13044=FACE_OUTER_BOUND('',#19223,.T.);
#13045=FACE_OUTER_BOUND('',#19225,.T.);
#13046=FACE_OUTER_BOUND('',#19227,.T.);
#13047=FACE_OUTER_BOUND('',#19229,.T.);
#13048=FACE_OUTER_BOUND('',#19230,.T.);
#13049=FACE_OUTER_BOUND('',#19231,.T.);
#13050=FACE_OUTER_BOUND('',#19232,.T.);
#13051=FACE_OUTER_BOUND('',#19233,.T.);
#13052=FACE_OUTER_BOUND('',#19234,.T.);
#13053=FACE_OUTER_BOUND('',#19235,.T.);
#13054=FACE_OUTER_BOUND('',#19236,.T.);
#13055=FACE_OUTER_BOUND('',#19237,.T.);
#13056=FACE_OUTER_BOUND('',#19238,.T.);
#13057=FACE_OUTER_BOUND('',#19239,.T.);
#13058=FACE_OUTER_BOUND('',#19240,.T.);
#13059=FACE_OUTER_BOUND('',#19242,.T.);
#13060=FACE_OUTER_BOUND('',#19244,.T.);
#13061=FACE_OUTER_BOUND('',#19246,.T.);
#13062=FACE_OUTER_BOUND('',#19248,.T.);
#13063=FACE_OUTER_BOUND('',#19250,.T.);
#13064=FACE_OUTER_BOUND('',#19251,.T.);
#13065=FACE_OUTER_BOUND('',#19252,.T.);
#13066=FACE_OUTER_BOUND('',#19253,.T.);
#13067=FACE_OUTER_BOUND('',#19254,.T.);
#13068=FACE_OUTER_BOUND('',#19255,.T.);
#13069=FACE_OUTER_BOUND('',#19256,.T.);
#13070=FACE_OUTER_BOUND('',#19257,.T.);
#13071=FACE_OUTER_BOUND('',#19258,.T.);
#13072=FACE_OUTER_BOUND('',#19259,.T.);
#13073=FACE_OUTER_BOUND('',#19260,.T.);
#13074=FACE_OUTER_BOUND('',#19261,.T.);
#13075=FACE_OUTER_BOUND('',#19262,.T.);
#13076=FACE_OUTER_BOUND('',#19263,.T.);
#13077=FACE_OUTER_BOUND('',#19264,.T.);
#13078=FACE_OUTER_BOUND('',#19265,.T.);
#13079=FACE_OUTER_BOUND('',#19266,.T.);
#13080=FACE_OUTER_BOUND('',#19267,.T.);
#13081=FACE_OUTER_BOUND('',#19268,.T.);
#13082=FACE_OUTER_BOUND('',#19270,.T.);
#13083=FACE_OUTER_BOUND('',#19271,.T.);
#13084=FACE_OUTER_BOUND('',#19272,.T.);
#13085=FACE_OUTER_BOUND('',#19273,.T.);
#13086=FACE_OUTER_BOUND('',#19274,.T.);
#13087=FACE_OUTER_BOUND('',#19275,.T.);
#13088=FACE_OUTER_BOUND('',#19276,.T.);
#13089=FACE_OUTER_BOUND('',#19277,.T.);
#13090=FACE_OUTER_BOUND('',#19278,.T.);
#13091=FACE_OUTER_BOUND('',#19279,.T.);
#13092=FACE_OUTER_BOUND('',#19280,.T.);
#13093=FACE_OUTER_BOUND('',#19281,.T.);
#13094=FACE_OUTER_BOUND('',#19282,.T.);
#13095=FACE_OUTER_BOUND('',#19283,.T.);
#13096=FACE_OUTER_BOUND('',#19284,.T.);
#13097=FACE_OUTER_BOUND('',#19285,.T.);
#13098=FACE_OUTER_BOUND('',#19286,.T.);
#13099=FACE_OUTER_BOUND('',#19287,.T.);
#13100=FACE_OUTER_BOUND('',#19288,.T.);
#13101=FACE_OUTER_BOUND('',#19289,.T.);
#13102=FACE_OUTER_BOUND('',#19290,.T.);
#13103=FACE_OUTER_BOUND('',#19291,.T.);
#13104=FACE_OUTER_BOUND('',#19292,.T.);
#13105=FACE_OUTER_BOUND('',#19293,.T.);
#13106=FACE_OUTER_BOUND('',#19294,.T.);
#13107=FACE_OUTER_BOUND('',#19295,.T.);
#13108=FACE_OUTER_BOUND('',#19296,.T.);
#13109=FACE_OUTER_BOUND('',#19297,.T.);
#13110=FACE_OUTER_BOUND('',#19298,.T.);
#13111=FACE_OUTER_BOUND('',#19299,.T.);
#13112=FACE_OUTER_BOUND('',#19300,.T.);
#13113=FACE_OUTER_BOUND('',#19301,.T.);
#13114=FACE_OUTER_BOUND('',#19302,.T.);
#13115=FACE_OUTER_BOUND('',#19303,.T.);
#13116=FACE_OUTER_BOUND('',#19304,.T.);
#13117=FACE_OUTER_BOUND('',#19306,.T.);
#13118=FACE_OUTER_BOUND('',#19307,.T.);
#13119=FACE_OUTER_BOUND('',#19308,.T.);
#13120=FACE_OUTER_BOUND('',#19309,.T.);
#13121=FACE_OUTER_BOUND('',#19310,.T.);
#13122=FACE_OUTER_BOUND('',#19311,.T.);
#13123=FACE_OUTER_BOUND('',#19312,.T.);
#13124=FACE_OUTER_BOUND('',#19313,.T.);
#13125=FACE_OUTER_BOUND('',#19314,.T.);
#13126=FACE_OUTER_BOUND('',#19315,.T.);
#13127=FACE_OUTER_BOUND('',#19316,.T.);
#13128=FACE_OUTER_BOUND('',#19317,.T.);
#13129=FACE_OUTER_BOUND('',#19318,.T.);
#13130=FACE_OUTER_BOUND('',#19319,.T.);
#13131=FACE_OUTER_BOUND('',#19320,.T.);
#13132=FACE_OUTER_BOUND('',#19321,.T.);
#13133=FACE_OUTER_BOUND('',#19322,.T.);
#13134=FACE_OUTER_BOUND('',#19323,.T.);
#13135=FACE_OUTER_BOUND('',#19324,.T.);
#13136=FACE_OUTER_BOUND('',#19325,.T.);
#13137=FACE_OUTER_BOUND('',#19326,.T.);
#13138=FACE_OUTER_BOUND('',#19328,.T.);
#13139=FACE_OUTER_BOUND('',#19329,.T.);
#13140=FACE_OUTER_BOUND('',#19330,.T.);
#13141=FACE_OUTER_BOUND('',#19332,.T.);
#13142=FACE_OUTER_BOUND('',#19334,.T.);
#13143=FACE_OUTER_BOUND('',#19336,.T.);
#13144=FACE_OUTER_BOUND('',#19337,.T.);
#13145=FACE_OUTER_BOUND('',#19338,.T.);
#13146=FACE_OUTER_BOUND('',#19339,.T.);
#13147=FACE_OUTER_BOUND('',#19340,.T.);
#13148=FACE_OUTER_BOUND('',#19341,.T.);
#13149=FACE_OUTER_BOUND('',#19342,.T.);
#13150=FACE_OUTER_BOUND('',#19343,.T.);
#13151=FACE_OUTER_BOUND('',#19344,.T.);
#13152=FACE_OUTER_BOUND('',#19345,.T.);
#13153=FACE_OUTER_BOUND('',#19346,.T.);
#13154=FACE_OUTER_BOUND('',#19347,.T.);
#13155=FACE_OUTER_BOUND('',#19348,.T.);
#13156=FACE_OUTER_BOUND('',#19349,.T.);
#13157=FACE_OUTER_BOUND('',#19350,.T.);
#13158=FACE_OUTER_BOUND('',#19351,.T.);
#13159=FACE_OUTER_BOUND('',#19352,.T.);
#13160=FACE_OUTER_BOUND('',#19353,.T.);
#13161=FACE_OUTER_BOUND('',#19354,.T.);
#13162=FACE_OUTER_BOUND('',#19355,.T.);
#13163=FACE_OUTER_BOUND('',#19356,.T.);
#13164=FACE_OUTER_BOUND('',#19357,.T.);
#13165=FACE_OUTER_BOUND('',#19358,.T.);
#13166=FACE_OUTER_BOUND('',#19359,.T.);
#13167=FACE_OUTER_BOUND('',#19365,.T.);
#13168=FACE_OUTER_BOUND('',#19367,.T.);
#13169=FACE_OUTER_BOUND('',#19369,.T.);
#13170=FACE_OUTER_BOUND('',#19371,.T.);
#13171=FACE_OUTER_BOUND('',#19373,.T.);
#13172=FACE_OUTER_BOUND('',#19375,.T.);
#13173=FACE_OUTER_BOUND('',#19376,.T.);
#13174=FACE_OUTER_BOUND('',#19377,.T.);
#13175=FACE_OUTER_BOUND('',#19378,.T.);
#13176=FACE_OUTER_BOUND('',#19379,.T.);
#13177=FACE_OUTER_BOUND('',#19380,.T.);
#13178=FACE_OUTER_BOUND('',#19381,.T.);
#13179=FACE_OUTER_BOUND('',#19382,.T.);
#13180=FACE_OUTER_BOUND('',#19383,.T.);
#13181=FACE_OUTER_BOUND('',#19384,.T.);
#13182=FACE_OUTER_BOUND('',#19385,.T.);
#13183=FACE_OUTER_BOUND('',#19386,.T.);
#13184=FACE_OUTER_BOUND('',#19387,.T.);
#13185=FACE_OUTER_BOUND('',#19388,.T.);
#13186=FACE_OUTER_BOUND('',#19389,.T.);
#13187=FACE_OUTER_BOUND('',#19390,.T.);
#13188=FACE_OUTER_BOUND('',#19391,.T.);
#13189=FACE_OUTER_BOUND('',#19397,.T.);
#13190=FACE_OUTER_BOUND('',#19398,.T.);
#13191=FACE_OUTER_BOUND('',#19400,.T.);
#13192=FACE_OUTER_BOUND('',#19402,.T.);
#13193=FACE_OUTER_BOUND('',#19404,.T.);
#13194=FACE_OUTER_BOUND('',#19406,.T.);
#13195=FACE_OUTER_BOUND('',#19407,.T.);
#13196=FACE_OUTER_BOUND('',#19408,.T.);
#13197=FACE_OUTER_BOUND('',#19409,.T.);
#13198=FACE_OUTER_BOUND('',#19411,.T.);
#13199=FACE_OUTER_BOUND('',#19412,.T.);
#13200=FACE_OUTER_BOUND('',#19413,.T.);
#13844=EDGE_LOOP('',(#60937,#60938,#60939,#60940,#60941));
#13845=EDGE_LOOP('',(#60942,#60943,#60944,#60945));
#13846=EDGE_LOOP('',(#60946,#60947,#60948,#60949));
#13847=EDGE_LOOP('',(#60950,#60951,#60952,#60953));
#13848=EDGE_LOOP('',(#60954,#60955,#60956,#60957,#60958));
#13849=EDGE_LOOP('',(#60959,#60960,#60961,#60962,#60963,#60964,#60965,#60966,
#60967,#60968,#60969));
#13850=EDGE_LOOP('',(#60970));
#13851=EDGE_LOOP('',(#60971));
#13852=EDGE_LOOP('',(#60972,#60973,#60974,#60975,#60976));
#13853=EDGE_LOOP('',(#60977,#60978,#60979,#60980,#60981,#60982));
#13854=EDGE_LOOP('',(#60983,#60984,#60985,#60986,#60987));
#13855=EDGE_LOOP('',(#60988,#60989,#60990,#60991));
#13856=EDGE_LOOP('',(#60992));
#13857=EDGE_LOOP('',(#60993));
#13858=EDGE_LOOP('',(#60994));
#13859=EDGE_LOOP('',(#60995,#60996,#60997,#60998));
#13860=EDGE_LOOP('',(#60999,#61000,#61001,#61002));
#13861=EDGE_LOOP('',(#61003,#61004,#61005,#61006));
#13862=EDGE_LOOP('',(#61007,#61008,#61009,#61010));
#13863=EDGE_LOOP('',(#61011,#61012,#61013,#61014));
#13864=EDGE_LOOP('',(#61015));
#13865=EDGE_LOOP('',(#61016,#61017,#61018,#61019,#61020,#61021));
#13866=EDGE_LOOP('',(#61022));
#13867=EDGE_LOOP('',(#61023,#61024,#61025,#61026));
#13868=EDGE_LOOP('',(#61027,#61028,#61029,#61030));
#13869=EDGE_LOOP('',(#61031,#61032,#61033,#61034));
#13870=EDGE_LOOP('',(#61035,#61036,#61037,#61038));
#13871=EDGE_LOOP('',(#61039,#61040,#61041,#61042));
#13872=EDGE_LOOP('',(#61043,#61044,#61045,#61046,#61047,#61048));
#13873=EDGE_LOOP('',(#61049,#61050,#61051,#61052,#61053,#61054));
#13874=EDGE_LOOP('',(#61055,#61056,#61057,#61058,#61059,#61060));
#13875=EDGE_LOOP('',(#61061,#61062,#61063,#61064,#61065,#61066));
#13876=EDGE_LOOP('',(#61067,#61068,#61069,#61070,#61071,#61072));
#13877=EDGE_LOOP('',(#61073,#61074,#61075,#61076,#61077,#61078));
#13878=EDGE_LOOP('',(#61079,#61080,#61081,#61082));
#13879=EDGE_LOOP('',(#61083,#61084,#61085,#61086));
#13880=EDGE_LOOP('',(#61087,#61088,#61089,#61090));
#13881=EDGE_LOOP('',(#61091,#61092,#61093,#61094));
#13882=EDGE_LOOP('',(#61095,#61096,#61097,#61098));
#13883=EDGE_LOOP('',(#61099,#61100,#61101,#61102));
#13884=EDGE_LOOP('',(#61103,#61104,#61105,#61106));
#13885=EDGE_LOOP('',(#61107));
#13886=EDGE_LOOP('',(#61108));
#13887=EDGE_LOOP('',(#61109));
#13888=EDGE_LOOP('',(#61110));
#13889=EDGE_LOOP('',(#61111,#61112,#61113,#61114));
#13890=EDGE_LOOP('',(#61115,#61116,#61117,#61118));
#13891=EDGE_LOOP('',(#61119));
#13892=EDGE_LOOP('',(#61120));
#13893=EDGE_LOOP('',(#61121));
#13894=EDGE_LOOP('',(#61122));
#13895=EDGE_LOOP('',(#61123,#61124,#61125,#61126));
#13896=EDGE_LOOP('',(#61127,#61128,#61129,#61130));
#13897=EDGE_LOOP('',(#61131));
#13898=EDGE_LOOP('',(#61132));
#13899=EDGE_LOOP('',(#61133));
#13900=EDGE_LOOP('',(#61134));
#13901=EDGE_LOOP('',(#61135,#61136,#61137,#61138));
#13902=EDGE_LOOP('',(#61139,#61140,#61141,#61142));
#13903=EDGE_LOOP('',(#61143));
#13904=EDGE_LOOP('',(#61144));
#13905=EDGE_LOOP('',(#61145));
#13906=EDGE_LOOP('',(#61146));
#13907=EDGE_LOOP('',(#61147,#61148,#61149,#61150,#61151));
#13908=EDGE_LOOP('',(#61152,#61153,#61154,#61155,#61156));
#13909=EDGE_LOOP('',(#61157,#61158,#61159,#61160,#61161));
#13910=EDGE_LOOP('',(#61162,#61163,#61164,#61165,#61166));
#13911=EDGE_LOOP('',(#61167));
#13912=EDGE_LOOP('',(#61168));
#13913=EDGE_LOOP('',(#61169));
#13914=EDGE_LOOP('',(#61170));
#13915=EDGE_LOOP('',(#61171,#61172,#61173,#61174,#61175));
#13916=EDGE_LOOP('',(#61176,#61177,#61178,#61179,#61180));
#13917=EDGE_LOOP('',(#61181,#61182,#61183,#61184,#61185));
#13918=EDGE_LOOP('',(#61186,#61187,#61188,#61189,#61190));
#13919=EDGE_LOOP('',(#61191));
#13920=EDGE_LOOP('',(#61192));
#13921=EDGE_LOOP('',(#61193));
#13922=EDGE_LOOP('',(#61194));
#13923=EDGE_LOOP('',(#61195,#61196,#61197,#61198));
#13924=EDGE_LOOP('',(#61199,#61200,#61201,#61202));
#13925=EDGE_LOOP('',(#61203));
#13926=EDGE_LOOP('',(#61204));
#13927=EDGE_LOOP('',(#61205));
#13928=EDGE_LOOP('',(#61206));
#13929=EDGE_LOOP('',(#61207,#61208,#61209,#61210));
#13930=EDGE_LOOP('',(#61211,#61212,#61213,#61214));
#13931=EDGE_LOOP('',(#61215,#61216,#61217,#61218));
#13932=EDGE_LOOP('',(#61219,#61220,#61221,#61222,#61223));
#13933=EDGE_LOOP('',(#61224,#61225,#61226,#61227,#61228));
#13934=EDGE_LOOP('',(#61229,#61230,#61231,#61232));
#13935=EDGE_LOOP('',(#61233,#61234,#61235,#61236,#61237));
#13936=EDGE_LOOP('',(#61238,#61239,#61240,#61241));
#13937=EDGE_LOOP('',(#61242,#61243,#61244,#61245));
#13938=EDGE_LOOP('',(#61246,#61247,#61248,#61249));
#13939=EDGE_LOOP('',(#61250,#61251,#61252,#61253,#61254,#61255,#61256,#61257,
#61258,#61259,#61260,#61261,#61262,#61263,#61264,#61265,#61266,#61267,#61268,
#61269,#61270,#61271,#61272,#61273,#61274,#61275,#61276,#61277,#61278,#61279,
#61280,#61281,#61282,#61283,#61284,#61285,#61286,#61287,#61288,#61289,#61290,
#61291,#61292,#61293,#61294,#61295,#61296,#61297,#61298,#61299,#61300,#61301,
#61302,#61303,#61304,#61305,#61306,#61307,#61308,#61309,#61310,#61311,#61312,
#61313,#61314,#61315,#61316,#61317,#61318,#61319,#61320,#61321,#61322,#61323,
#61324,#61325,#61326,#61327,#61328,#61329,#61330,#61331,#61332,#61333,#61334,
#61335,#61336,#61337,#61338,#61339,#61340,#61341,#61342,#61343,#61344,#61345,
#61346,#61347,#61348,#61349,#61350,#61351,#61352,#61353,#61354,#61355,#61356,
#61357,#61358,#61359,#61360,#61361,#61362,#61363,#61364,#61365,#61366,#61367,
#61368,#61369,#61370,#61371,#61372,#61373,#61374,#61375,#61376,#61377,#61378,
#61379,#61380,#61381,#61382,#61383,#61384,#61385,#61386,#61387,#61388,#61389,
#61390,#61391,#61392,#61393,#61394,#61395,#61396,#61397,#61398,#61399,#61400,
#61401,#61402,#61403,#61404,#61405,#61406,#61407,#61408,#61409,#61410,#61411,
#61412,#61413,#61414,#61415,#61416,#61417,#61418,#61419,#61420,#61421,#61422,
#61423,#61424,#61425,#61426,#61427,#61428,#61429,#61430,#61431,#61432,#61433,
#61434,#61435,#61436,#61437,#61438,#61439,#61440,#61441,#61442,#61443,#61444,
#61445,#61446,#61447,#61448,#61449,#61450,#61451,#61452,#61453,#61454,#61455,
#61456,#61457,#61458,#61459,#61460,#61461,#61462,#61463,#61464,#61465,#61466,
#61467,#61468,#61469,#61470,#61471,#61472,#61473,#61474,#61475,#61476,#61477,
#61478,#61479,#61480,#61481,#61482,#61483,#61484,#61485,#61486,#61487,#61488,
#61489,#61490,#61491,#61492,#61493,#61494,#61495,#61496,#61497,#61498,#61499,
#61500,#61501,#61502,#61503,#61504,#61505,#61506,#61507,#61508,#61509,#61510,
#61511,#61512,#61513,#61514,#61515,#61516,#61517,#61518,#61519,#61520,#61521,
#61522,#61523,#61524,#61525,#61526,#61527,#61528,#61529,#61530,#61531,#61532,
#61533,#61534,#61535,#61536,#61537,#61538,#61539,#61540,#61541,#61542,#61543,
#61544,#61545,#61546,#61547,#61548,#61549,#61550,#61551,#61552,#61553,#61554,
#61555,#61556,#61557,#61558,#61559,#61560,#61561,#61562,#61563,#61564,#61565,
#61566,#61567,#61568,#61569,#61570,#61571,#61572,#61573,#61574,#61575,#61576,
#61577,#61578,#61579,#61580,#61581,#61582,#61583,#61584,#61585,#61586,#61587,
#61588,#61589,#61590,#61591,#61592,#61593,#61594,#61595,#61596,#61597,#61598,
#61599,#61600,#61601,#61602,#61603,#61604,#61605,#61606,#61607,#61608,#61609,
#61610,#61611,#61612,#61613,#61614));
#13940=EDGE_LOOP('',(#61615,#61616,#61617,#61618,#61619,#61620,#61621,#61622,
#61623,#61624,#61625,#61626,#61627,#61628,#61629,#61630,#61631,#61632,#61633,
#61634,#61635,#61636,#61637,#61638,#61639,#61640,#61641,#61642,#61643,#61644,
#61645,#61646,#61647,#61648,#61649,#61650,#61651,#61652,#61653,#61654,#61655,
#61656,#61657,#61658,#61659,#61660,#61661,#61662,#61663,#61664,#61665,#61666,
#61667,#61668,#61669,#61670,#61671,#61672,#61673,#61674,#61675,#61676,#61677,
#61678,#61679,#61680,#61681,#61682,#61683,#61684,#61685,#61686,#61687,#61688,
#61689,#61690,#61691,#61692,#61693,#61694,#61695,#61696,#61697,#61698,#61699,
#61700,#61701,#61702,#61703,#61704,#61705,#61706,#61707,#61708,#61709,#61710,
#61711,#61712,#61713,#61714,#61715,#61716,#61717,#61718,#61719,#61720,#61721,
#61722,#61723,#61724,#61725,#61726,#61727,#61728,#61729,#61730,#61731,#61732,
#61733,#61734,#61735,#61736,#61737,#61738,#61739,#61740,#61741,#61742,#61743,
#61744,#61745,#61746,#61747,#61748,#61749,#61750,#61751,#61752,#61753,#61754,
#61755,#61756,#61757,#61758,#61759,#61760,#61761,#61762,#61763,#61764,#61765,
#61766,#61767,#61768,#61769,#61770,#61771,#61772,#61773,#61774,#61775,#61776,
#61777,#61778,#61779,#61780,#61781,#61782,#61783,#61784,#61785,#61786,#61787,
#61788,#61789,#61790,#61791,#61792,#61793,#61794,#61795,#61796,#61797,#61798,
#61799,#61800,#61801,#61802,#61803,#61804,#61805,#61806,#61807,#61808,#61809,
#61810,#61811,#61812,#61813,#61814,#61815,#61816,#61817,#61818,#61819,#61820,
#61821,#61822,#61823,#61824,#61825,#61826,#61827,#61828,#61829,#61830,#61831,
#61832,#61833,#61834,#61835,#61836,#61837,#61838,#61839,#61840,#61841,#61842,
#61843,#61844,#61845,#61846,#61847,#61848,#61849,#61850,#61851,#61852,#61853,
#61854,#61855,#61856,#61857,#61858,#61859,#61860,#61861,#61862,#61863,#61864,
#61865,#61866,#61867,#61868,#61869,#61870,#61871,#61872,#61873,#61874,#61875,
#61876,#61877,#61878,#61879,#61880,#61881,#61882,#61883,#61884,#61885,#61886,
#61887,#61888,#61889,#61890,#61891,#61892,#61893,#61894,#61895,#61896,#61897,
#61898,#61899,#61900,#61901,#61902,#61903,#61904,#61905,#61906,#61907,#61908,
#61909,#61910,#61911,#61912,#61913,#61914,#61915,#61916,#61917,#61918,#61919,
#61920,#61921,#61922,#61923,#61924,#61925,#61926,#61927,#61928,#61929,#61930,
#61931,#61932,#61933,#61934,#61935,#61936,#61937,#61938,#61939,#61940,#61941,
#61942,#61943,#61944,#61945,#61946,#61947,#61948,#61949,#61950,#61951,#61952,
#61953,#61954,#61955,#61956,#61957,#61958,#61959,#61960,#61961,#61962,#61963,
#61964,#61965,#61966,#61967,#61968,#61969,#61970,#61971,#61972,#61973,#61974,
#61975,#61976,#61977,#61978));
#13941=EDGE_LOOP('',(#61979,#61980,#61981,#61982,#61983,#61984));
#13942=EDGE_LOOP('',(#61985,#61986,#61987,#61988,#61989));
#13943=EDGE_LOOP('',(#61990,#61991,#61992,#61993,#61994,#61995));
#13944=EDGE_LOOP('',(#61996,#61997,#61998,#61999));
#13945=EDGE_LOOP('',(#62000,#62001,#62002,#62003));
#13946=EDGE_LOOP('',(#62004,#62005,#62006,#62007,#62008,#62009));
#13947=EDGE_LOOP('',(#62010,#62011,#62012,#62013));
#13948=EDGE_LOOP('',(#62014,#62015,#62016,#62017));
#13949=EDGE_LOOP('',(#62018,#62019,#62020,#62021));
#13950=EDGE_LOOP('',(#62022,#62023,#62024,#62025));
#13951=EDGE_LOOP('',(#62026,#62027,#62028,#62029));
#13952=EDGE_LOOP('',(#62030,#62031,#62032,#62033,#62034,#62035));
#13953=EDGE_LOOP('',(#62036,#62037,#62038,#62039));
#13954=EDGE_LOOP('',(#62040,#62041,#62042,#62043));
#13955=EDGE_LOOP('',(#62044,#62045,#62046,#62047,#62048,#62049));
#13956=EDGE_LOOP('',(#62050,#62051,#62052,#62053));
#13957=EDGE_LOOP('',(#62054,#62055,#62056,#62057));
#13958=EDGE_LOOP('',(#62058,#62059,#62060,#62061));
#13959=EDGE_LOOP('',(#62062,#62063,#62064,#62065));
#13960=EDGE_LOOP('',(#62066,#62067,#62068,#62069));
#13961=EDGE_LOOP('',(#62070,#62071,#62072,#62073,#62074,#62075));
#13962=EDGE_LOOP('',(#62076,#62077,#62078,#62079));
#13963=EDGE_LOOP('',(#62080,#62081,#62082,#62083));
#13964=EDGE_LOOP('',(#62084,#62085,#62086,#62087,#62088,#62089));
#13965=EDGE_LOOP('',(#62090,#62091,#62092,#62093));
#13966=EDGE_LOOP('',(#62094,#62095,#62096,#62097));
#13967=EDGE_LOOP('',(#62098,#62099,#62100,#62101));
#13968=EDGE_LOOP('',(#62102,#62103,#62104,#62105));
#13969=EDGE_LOOP('',(#62106,#62107,#62108,#62109));
#13970=EDGE_LOOP('',(#62110,#62111,#62112,#62113,#62114,#62115));
#13971=EDGE_LOOP('',(#62116,#62117,#62118,#62119));
#13972=EDGE_LOOP('',(#62120,#62121,#62122,#62123));
#13973=EDGE_LOOP('',(#62124,#62125,#62126,#62127,#62128,#62129));
#13974=EDGE_LOOP('',(#62130,#62131,#62132,#62133));
#13975=EDGE_LOOP('',(#62134,#62135,#62136,#62137));
#13976=EDGE_LOOP('',(#62138,#62139,#62140,#62141));
#13977=EDGE_LOOP('',(#62142,#62143,#62144,#62145));
#13978=EDGE_LOOP('',(#62146,#62147,#62148,#62149));
#13979=EDGE_LOOP('',(#62150,#62151,#62152,#62153,#62154,#62155));
#13980=EDGE_LOOP('',(#62156,#62157,#62158,#62159));
#13981=EDGE_LOOP('',(#62160,#62161,#62162,#62163));
#13982=EDGE_LOOP('',(#62164,#62165,#62166,#62167,#62168,#62169));
#13983=EDGE_LOOP('',(#62170,#62171,#62172,#62173));
#13984=EDGE_LOOP('',(#62174,#62175,#62176,#62177));
#13985=EDGE_LOOP('',(#62178,#62179,#62180,#62181));
#13986=EDGE_LOOP('',(#62182,#62183,#62184,#62185));
#13987=EDGE_LOOP('',(#62186,#62187,#62188,#62189));
#13988=EDGE_LOOP('',(#62190,#62191,#62192,#62193,#62194,#62195));
#13989=EDGE_LOOP('',(#62196,#62197,#62198,#62199));
#13990=EDGE_LOOP('',(#62200,#62201,#62202,#62203));
#13991=EDGE_LOOP('',(#62204,#62205,#62206,#62207,#62208,#62209));
#13992=EDGE_LOOP('',(#62210,#62211,#62212,#62213));
#13993=EDGE_LOOP('',(#62214,#62215,#62216,#62217));
#13994=EDGE_LOOP('',(#62218,#62219,#62220,#62221));
#13995=EDGE_LOOP('',(#62222,#62223,#62224,#62225));
#13996=EDGE_LOOP('',(#62226,#62227,#62228,#62229));
#13997=EDGE_LOOP('',(#62230,#62231,#62232,#62233,#62234,#62235));
#13998=EDGE_LOOP('',(#62236,#62237,#62238,#62239));
#13999=EDGE_LOOP('',(#62240,#62241,#62242,#62243));
#14000=EDGE_LOOP('',(#62244,#62245,#62246,#62247,#62248,#62249));
#14001=EDGE_LOOP('',(#62250,#62251,#62252,#62253));
#14002=EDGE_LOOP('',(#62254,#62255,#62256,#62257));
#14003=EDGE_LOOP('',(#62258,#62259,#62260,#62261));
#14004=EDGE_LOOP('',(#62262,#62263,#62264,#62265));
#14005=EDGE_LOOP('',(#62266,#62267,#62268,#62269));
#14006=EDGE_LOOP('',(#62270,#62271,#62272,#62273,#62274,#62275));
#14007=EDGE_LOOP('',(#62276,#62277,#62278,#62279));
#14008=EDGE_LOOP('',(#62280,#62281,#62282,#62283));
#14009=EDGE_LOOP('',(#62284,#62285,#62286,#62287,#62288,#62289));
#14010=EDGE_LOOP('',(#62290,#62291,#62292,#62293));
#14011=EDGE_LOOP('',(#62294,#62295,#62296,#62297));
#14012=EDGE_LOOP('',(#62298,#62299,#62300,#62301));
#14013=EDGE_LOOP('',(#62302,#62303,#62304,#62305));
#14014=EDGE_LOOP('',(#62306,#62307,#62308,#62309));
#14015=EDGE_LOOP('',(#62310,#62311,#62312,#62313,#62314,#62315));
#14016=EDGE_LOOP('',(#62316,#62317,#62318,#62319));
#14017=EDGE_LOOP('',(#62320,#62321,#62322,#62323));
#14018=EDGE_LOOP('',(#62324,#62325,#62326,#62327,#62328,#62329));
#14019=EDGE_LOOP('',(#62330,#62331,#62332,#62333));
#14020=EDGE_LOOP('',(#62334,#62335,#62336,#62337));
#14021=EDGE_LOOP('',(#62338,#62339,#62340,#62341));
#14022=EDGE_LOOP('',(#62342,#62343,#62344,#62345));
#14023=EDGE_LOOP('',(#62346,#62347,#62348,#62349));
#14024=EDGE_LOOP('',(#62350,#62351,#62352,#62353,#62354,#62355));
#14025=EDGE_LOOP('',(#62356,#62357,#62358,#62359));
#14026=EDGE_LOOP('',(#62360,#62361,#62362,#62363));
#14027=EDGE_LOOP('',(#62364,#62365,#62366,#62367,#62368,#62369));
#14028=EDGE_LOOP('',(#62370,#62371,#62372,#62373));
#14029=EDGE_LOOP('',(#62374,#62375,#62376,#62377));
#14030=EDGE_LOOP('',(#62378,#62379,#62380,#62381));
#14031=EDGE_LOOP('',(#62382,#62383,#62384,#62385));
#14032=EDGE_LOOP('',(#62386,#62387,#62388,#62389));
#14033=EDGE_LOOP('',(#62390,#62391,#62392,#62393,#62394,#62395));
#14034=EDGE_LOOP('',(#62396,#62397,#62398,#62399));
#14035=EDGE_LOOP('',(#62400,#62401,#62402,#62403));
#14036=EDGE_LOOP('',(#62404,#62405,#62406,#62407,#62408,#62409));
#14037=EDGE_LOOP('',(#62410,#62411,#62412,#62413));
#14038=EDGE_LOOP('',(#62414,#62415,#62416,#62417));
#14039=EDGE_LOOP('',(#62418,#62419,#62420,#62421));
#14040=EDGE_LOOP('',(#62422,#62423,#62424,#62425));
#14041=EDGE_LOOP('',(#62426,#62427,#62428,#62429));
#14042=EDGE_LOOP('',(#62430,#62431,#62432,#62433,#62434,#62435));
#14043=EDGE_LOOP('',(#62436,#62437,#62438,#62439));
#14044=EDGE_LOOP('',(#62440,#62441,#62442,#62443));
#14045=EDGE_LOOP('',(#62444,#62445,#62446,#62447,#62448,#62449));
#14046=EDGE_LOOP('',(#62450,#62451,#62452,#62453));
#14047=EDGE_LOOP('',(#62454,#62455,#62456,#62457));
#14048=EDGE_LOOP('',(#62458,#62459,#62460,#62461));
#14049=EDGE_LOOP('',(#62462,#62463,#62464,#62465));
#14050=EDGE_LOOP('',(#62466,#62467,#62468,#62469));
#14051=EDGE_LOOP('',(#62470,#62471,#62472,#62473,#62474,#62475));
#14052=EDGE_LOOP('',(#62476,#62477,#62478,#62479));
#14053=EDGE_LOOP('',(#62480,#62481,#62482,#62483));
#14054=EDGE_LOOP('',(#62484,#62485,#62486,#62487,#62488,#62489));
#14055=EDGE_LOOP('',(#62490,#62491,#62492,#62493));
#14056=EDGE_LOOP('',(#62494,#62495,#62496,#62497));
#14057=EDGE_LOOP('',(#62498,#62499,#62500,#62501));
#14058=EDGE_LOOP('',(#62502,#62503,#62504,#62505));
#14059=EDGE_LOOP('',(#62506,#62507,#62508,#62509));
#14060=EDGE_LOOP('',(#62510,#62511,#62512,#62513,#62514,#62515));
#14061=EDGE_LOOP('',(#62516,#62517,#62518,#62519));
#14062=EDGE_LOOP('',(#62520,#62521,#62522,#62523));
#14063=EDGE_LOOP('',(#62524,#62525,#62526,#62527,#62528,#62529));
#14064=EDGE_LOOP('',(#62530,#62531,#62532,#62533));
#14065=EDGE_LOOP('',(#62534,#62535,#62536,#62537));
#14066=EDGE_LOOP('',(#62538,#62539,#62540,#62541));
#14067=EDGE_LOOP('',(#62542,#62543,#62544,#62545));
#14068=EDGE_LOOP('',(#62546,#62547,#62548,#62549));
#14069=EDGE_LOOP('',(#62550,#62551,#62552,#62553,#62554,#62555));
#14070=EDGE_LOOP('',(#62556,#62557,#62558,#62559));
#14071=EDGE_LOOP('',(#62560,#62561,#62562,#62563));
#14072=EDGE_LOOP('',(#62564,#62565,#62566,#62567,#62568,#62569));
#14073=EDGE_LOOP('',(#62570,#62571,#62572,#62573));
#14074=EDGE_LOOP('',(#62574,#62575,#62576,#62577));
#14075=EDGE_LOOP('',(#62578,#62579,#62580,#62581));
#14076=EDGE_LOOP('',(#62582,#62583,#62584,#62585));
#14077=EDGE_LOOP('',(#62586,#62587,#62588,#62589));
#14078=EDGE_LOOP('',(#62590,#62591,#62592,#62593,#62594,#62595));
#14079=EDGE_LOOP('',(#62596,#62597,#62598,#62599));
#14080=EDGE_LOOP('',(#62600,#62601,#62602,#62603));
#14081=EDGE_LOOP('',(#62604,#62605,#62606,#62607,#62608,#62609));
#14082=EDGE_LOOP('',(#62610,#62611,#62612,#62613));
#14083=EDGE_LOOP('',(#62614,#62615,#62616,#62617));
#14084=EDGE_LOOP('',(#62618,#62619,#62620,#62621));
#14085=EDGE_LOOP('',(#62622,#62623,#62624,#62625));
#14086=EDGE_LOOP('',(#62626,#62627,#62628,#62629));
#14087=EDGE_LOOP('',(#62630,#62631,#62632,#62633,#62634,#62635));
#14088=EDGE_LOOP('',(#62636,#62637,#62638,#62639));
#14089=EDGE_LOOP('',(#62640,#62641,#62642,#62643));
#14090=EDGE_LOOP('',(#62644,#62645,#62646,#62647,#62648,#62649));
#14091=EDGE_LOOP('',(#62650,#62651,#62652,#62653));
#14092=EDGE_LOOP('',(#62654,#62655,#62656,#62657));
#14093=EDGE_LOOP('',(#62658,#62659,#62660,#62661));
#14094=EDGE_LOOP('',(#62662,#62663,#62664,#62665));
#14095=EDGE_LOOP('',(#62666,#62667,#62668,#62669));
#14096=EDGE_LOOP('',(#62670,#62671,#62672,#62673,#62674,#62675));
#14097=EDGE_LOOP('',(#62676,#62677,#62678,#62679));
#14098=EDGE_LOOP('',(#62680,#62681,#62682,#62683));
#14099=EDGE_LOOP('',(#62684,#62685,#62686,#62687,#62688,#62689));
#14100=EDGE_LOOP('',(#62690,#62691,#62692,#62693));
#14101=EDGE_LOOP('',(#62694,#62695,#62696,#62697));
#14102=EDGE_LOOP('',(#62698,#62699,#62700,#62701));
#14103=EDGE_LOOP('',(#62702,#62703,#62704,#62705));
#14104=EDGE_LOOP('',(#62706,#62707,#62708,#62709));
#14105=EDGE_LOOP('',(#62710,#62711,#62712,#62713,#62714,#62715));
#14106=EDGE_LOOP('',(#62716,#62717,#62718,#62719));
#14107=EDGE_LOOP('',(#62720,#62721,#62722,#62723));
#14108=EDGE_LOOP('',(#62724,#62725,#62726,#62727,#62728,#62729));
#14109=EDGE_LOOP('',(#62730,#62731,#62732,#62733));
#14110=EDGE_LOOP('',(#62734,#62735,#62736,#62737));
#14111=EDGE_LOOP('',(#62738,#62739,#62740,#62741));
#14112=EDGE_LOOP('',(#62742,#62743,#62744,#62745));
#14113=EDGE_LOOP('',(#62746,#62747,#62748,#62749));
#14114=EDGE_LOOP('',(#62750,#62751,#62752,#62753,#62754,#62755));
#14115=EDGE_LOOP('',(#62756,#62757,#62758,#62759));
#14116=EDGE_LOOP('',(#62760,#62761,#62762,#62763));
#14117=EDGE_LOOP('',(#62764,#62765,#62766,#62767,#62768,#62769));
#14118=EDGE_LOOP('',(#62770,#62771,#62772,#62773));
#14119=EDGE_LOOP('',(#62774,#62775,#62776,#62777));
#14120=EDGE_LOOP('',(#62778,#62779,#62780,#62781));
#14121=EDGE_LOOP('',(#62782,#62783,#62784,#62785));
#14122=EDGE_LOOP('',(#62786,#62787,#62788,#62789));
#14123=EDGE_LOOP('',(#62790,#62791,#62792,#62793,#62794,#62795));
#14124=EDGE_LOOP('',(#62796,#62797,#62798,#62799));
#14125=EDGE_LOOP('',(#62800,#62801,#62802,#62803));
#14126=EDGE_LOOP('',(#62804,#62805,#62806,#62807,#62808,#62809));
#14127=EDGE_LOOP('',(#62810,#62811,#62812,#62813));
#14128=EDGE_LOOP('',(#62814,#62815,#62816,#62817));
#14129=EDGE_LOOP('',(#62818,#62819,#62820,#62821));
#14130=EDGE_LOOP('',(#62822,#62823,#62824,#62825));
#14131=EDGE_LOOP('',(#62826,#62827,#62828,#62829));
#14132=EDGE_LOOP('',(#62830,#62831,#62832,#62833,#62834,#62835));
#14133=EDGE_LOOP('',(#62836,#62837,#62838,#62839));
#14134=EDGE_LOOP('',(#62840,#62841,#62842,#62843));
#14135=EDGE_LOOP('',(#62844,#62845,#62846,#62847,#62848,#62849));
#14136=EDGE_LOOP('',(#62850,#62851,#62852,#62853));
#14137=EDGE_LOOP('',(#62854,#62855,#62856,#62857));
#14138=EDGE_LOOP('',(#62858,#62859,#62860,#62861));
#14139=EDGE_LOOP('',(#62862,#62863,#62864,#62865));
#14140=EDGE_LOOP('',(#62866,#62867,#62868,#62869));
#14141=EDGE_LOOP('',(#62870,#62871,#62872,#62873,#62874,#62875));
#14142=EDGE_LOOP('',(#62876,#62877,#62878,#62879));
#14143=EDGE_LOOP('',(#62880,#62881,#62882,#62883));
#14144=EDGE_LOOP('',(#62884,#62885,#62886,#62887,#62888,#62889));
#14145=EDGE_LOOP('',(#62890,#62891,#62892,#62893));
#14146=EDGE_LOOP('',(#62894,#62895,#62896,#62897));
#14147=EDGE_LOOP('',(#62898,#62899,#62900,#62901));
#14148=EDGE_LOOP('',(#62902,#62903,#62904,#62905));
#14149=EDGE_LOOP('',(#62906,#62907,#62908,#62909));
#14150=EDGE_LOOP('',(#62910,#62911,#62912,#62913,#62914,#62915));
#14151=EDGE_LOOP('',(#62916,#62917,#62918,#62919));
#14152=EDGE_LOOP('',(#62920,#62921,#62922,#62923));
#14153=EDGE_LOOP('',(#62924,#62925,#62926,#62927,#62928,#62929));
#14154=EDGE_LOOP('',(#62930,#62931,#62932,#62933));
#14155=EDGE_LOOP('',(#62934,#62935,#62936,#62937));
#14156=EDGE_LOOP('',(#62938,#62939,#62940,#62941));
#14157=EDGE_LOOP('',(#62942,#62943,#62944,#62945));
#14158=EDGE_LOOP('',(#62946,#62947,#62948,#62949));
#14159=EDGE_LOOP('',(#62950,#62951,#62952,#62953,#62954,#62955));
#14160=EDGE_LOOP('',(#62956,#62957,#62958,#62959));
#14161=EDGE_LOOP('',(#62960,#62961,#62962,#62963));
#14162=EDGE_LOOP('',(#62964,#62965,#62966,#62967,#62968,#62969));
#14163=EDGE_LOOP('',(#62970,#62971,#62972,#62973));
#14164=EDGE_LOOP('',(#62974,#62975,#62976,#62977));
#14165=EDGE_LOOP('',(#62978,#62979,#62980,#62981));
#14166=EDGE_LOOP('',(#62982,#62983,#62984,#62985));
#14167=EDGE_LOOP('',(#62986,#62987,#62988,#62989));
#14168=EDGE_LOOP('',(#62990,#62991,#62992,#62993,#62994,#62995));
#14169=EDGE_LOOP('',(#62996,#62997,#62998,#62999));
#14170=EDGE_LOOP('',(#63000,#63001,#63002,#63003));
#14171=EDGE_LOOP('',(#63004,#63005,#63006,#63007,#63008,#63009));
#14172=EDGE_LOOP('',(#63010,#63011,#63012,#63013));
#14173=EDGE_LOOP('',(#63014,#63015,#63016,#63017));
#14174=EDGE_LOOP('',(#63018,#63019,#63020,#63021));
#14175=EDGE_LOOP('',(#63022,#63023,#63024,#63025));
#14176=EDGE_LOOP('',(#63026,#63027,#63028,#63029));
#14177=EDGE_LOOP('',(#63030,#63031,#63032,#63033,#63034,#63035));
#14178=EDGE_LOOP('',(#63036,#63037,#63038,#63039));
#14179=EDGE_LOOP('',(#63040,#63041,#63042,#63043));
#14180=EDGE_LOOP('',(#63044,#63045,#63046,#63047,#63048,#63049));
#14181=EDGE_LOOP('',(#63050,#63051,#63052,#63053));
#14182=EDGE_LOOP('',(#63054,#63055,#63056,#63057));
#14183=EDGE_LOOP('',(#63058,#63059,#63060,#63061));
#14184=EDGE_LOOP('',(#63062,#63063,#63064,#63065));
#14185=EDGE_LOOP('',(#63066,#63067,#63068,#63069));
#14186=EDGE_LOOP('',(#63070,#63071,#63072,#63073,#63074,#63075));
#14187=EDGE_LOOP('',(#63076,#63077,#63078,#63079));
#14188=EDGE_LOOP('',(#63080,#63081,#63082,#63083));
#14189=EDGE_LOOP('',(#63084,#63085,#63086,#63087,#63088,#63089));
#14190=EDGE_LOOP('',(#63090,#63091,#63092,#63093));
#14191=EDGE_LOOP('',(#63094,#63095,#63096,#63097));
#14192=EDGE_LOOP('',(#63098,#63099,#63100,#63101));
#14193=EDGE_LOOP('',(#63102,#63103,#63104,#63105));
#14194=EDGE_LOOP('',(#63106,#63107,#63108,#63109));
#14195=EDGE_LOOP('',(#63110,#63111,#63112,#63113,#63114,#63115));
#14196=EDGE_LOOP('',(#63116,#63117,#63118,#63119));
#14197=EDGE_LOOP('',(#63120,#63121,#63122,#63123));
#14198=EDGE_LOOP('',(#63124,#63125,#63126,#63127,#63128,#63129));
#14199=EDGE_LOOP('',(#63130,#63131,#63132,#63133));
#14200=EDGE_LOOP('',(#63134,#63135,#63136,#63137));
#14201=EDGE_LOOP('',(#63138,#63139,#63140,#63141));
#14202=EDGE_LOOP('',(#63142,#63143,#63144,#63145));
#14203=EDGE_LOOP('',(#63146,#63147,#63148,#63149));
#14204=EDGE_LOOP('',(#63150,#63151,#63152,#63153,#63154,#63155));
#14205=EDGE_LOOP('',(#63156,#63157,#63158,#63159));
#14206=EDGE_LOOP('',(#63160,#63161,#63162,#63163));
#14207=EDGE_LOOP('',(#63164,#63165,#63166,#63167,#63168,#63169));
#14208=EDGE_LOOP('',(#63170,#63171,#63172,#63173));
#14209=EDGE_LOOP('',(#63174,#63175,#63176,#63177));
#14210=EDGE_LOOP('',(#63178,#63179,#63180,#63181));
#14211=EDGE_LOOP('',(#63182,#63183,#63184,#63185));
#14212=EDGE_LOOP('',(#63186,#63187,#63188,#63189));
#14213=EDGE_LOOP('',(#63190,#63191,#63192,#63193,#63194,#63195));
#14214=EDGE_LOOP('',(#63196,#63197,#63198,#63199));
#14215=EDGE_LOOP('',(#63200,#63201,#63202,#63203));
#14216=EDGE_LOOP('',(#63204,#63205,#63206,#63207,#63208,#63209));
#14217=EDGE_LOOP('',(#63210,#63211,#63212,#63213));
#14218=EDGE_LOOP('',(#63214,#63215,#63216,#63217));
#14219=EDGE_LOOP('',(#63218,#63219,#63220,#63221));
#14220=EDGE_LOOP('',(#63222,#63223,#63224,#63225));
#14221=EDGE_LOOP('',(#63226,#63227,#63228,#63229));
#14222=EDGE_LOOP('',(#63230,#63231,#63232,#63233,#63234,#63235));
#14223=EDGE_LOOP('',(#63236,#63237,#63238,#63239));
#14224=EDGE_LOOP('',(#63240,#63241,#63242,#63243));
#14225=EDGE_LOOP('',(#63244,#63245,#63246,#63247,#63248,#63249));
#14226=EDGE_LOOP('',(#63250,#63251,#63252,#63253));
#14227=EDGE_LOOP('',(#63254,#63255,#63256,#63257));
#14228=EDGE_LOOP('',(#63258,#63259,#63260,#63261));
#14229=EDGE_LOOP('',(#63262,#63263,#63264,#63265));
#14230=EDGE_LOOP('',(#63266,#63267,#63268,#63269));
#14231=EDGE_LOOP('',(#63270,#63271,#63272,#63273,#63274,#63275));
#14232=EDGE_LOOP('',(#63276,#63277,#63278,#63279));
#14233=EDGE_LOOP('',(#63280,#63281,#63282,#63283));
#14234=EDGE_LOOP('',(#63284,#63285,#63286,#63287,#63288,#63289));
#14235=EDGE_LOOP('',(#63290,#63291,#63292,#63293));
#14236=EDGE_LOOP('',(#63294,#63295,#63296,#63297));
#14237=EDGE_LOOP('',(#63298,#63299,#63300,#63301));
#14238=EDGE_LOOP('',(#63302,#63303,#63304,#63305));
#14239=EDGE_LOOP('',(#63306,#63307,#63308,#63309));
#14240=EDGE_LOOP('',(#63310,#63311,#63312,#63313,#63314,#63315));
#14241=EDGE_LOOP('',(#63316,#63317,#63318,#63319));
#14242=EDGE_LOOP('',(#63320,#63321,#63322,#63323));
#14243=EDGE_LOOP('',(#63324,#63325,#63326,#63327,#63328,#63329));
#14244=EDGE_LOOP('',(#63330,#63331,#63332,#63333));
#14245=EDGE_LOOP('',(#63334,#63335,#63336,#63337));
#14246=EDGE_LOOP('',(#63338,#63339,#63340,#63341));
#14247=EDGE_LOOP('',(#63342,#63343,#63344,#63345));
#14248=EDGE_LOOP('',(#63346,#63347,#63348,#63349));
#14249=EDGE_LOOP('',(#63350,#63351,#63352,#63353,#63354,#63355));
#14250=EDGE_LOOP('',(#63356,#63357,#63358,#63359));
#14251=EDGE_LOOP('',(#63360,#63361,#63362,#63363));
#14252=EDGE_LOOP('',(#63364,#63365,#63366,#63367,#63368,#63369));
#14253=EDGE_LOOP('',(#63370,#63371,#63372,#63373));
#14254=EDGE_LOOP('',(#63374,#63375,#63376,#63377));
#14255=EDGE_LOOP('',(#63378,#63379,#63380,#63381));
#14256=EDGE_LOOP('',(#63382,#63383,#63384,#63385));
#14257=EDGE_LOOP('',(#63386,#63387,#63388,#63389));
#14258=EDGE_LOOP('',(#63390,#63391,#63392,#63393,#63394,#63395));
#14259=EDGE_LOOP('',(#63396,#63397,#63398,#63399));
#14260=EDGE_LOOP('',(#63400,#63401,#63402,#63403));
#14261=EDGE_LOOP('',(#63404,#63405,#63406,#63407,#63408,#63409));
#14262=EDGE_LOOP('',(#63410,#63411,#63412,#63413));
#14263=EDGE_LOOP('',(#63414,#63415,#63416,#63417));
#14264=EDGE_LOOP('',(#63418,#63419,#63420,#63421));
#14265=EDGE_LOOP('',(#63422,#63423,#63424,#63425));
#14266=EDGE_LOOP('',(#63426,#63427,#63428,#63429));
#14267=EDGE_LOOP('',(#63430,#63431,#63432,#63433,#63434,#63435));
#14268=EDGE_LOOP('',(#63436,#63437,#63438,#63439));
#14269=EDGE_LOOP('',(#63440,#63441,#63442,#63443));
#14270=EDGE_LOOP('',(#63444,#63445,#63446,#63447,#63448,#63449));
#14271=EDGE_LOOP('',(#63450,#63451,#63452,#63453));
#14272=EDGE_LOOP('',(#63454,#63455,#63456,#63457));
#14273=EDGE_LOOP('',(#63458,#63459,#63460,#63461));
#14274=EDGE_LOOP('',(#63462,#63463,#63464,#63465));
#14275=EDGE_LOOP('',(#63466,#63467,#63468,#63469));
#14276=EDGE_LOOP('',(#63470,#63471,#63472,#63473,#63474,#63475));
#14277=EDGE_LOOP('',(#63476,#63477,#63478,#63479));
#14278=EDGE_LOOP('',(#63480,#63481,#63482,#63483));
#14279=EDGE_LOOP('',(#63484,#63485,#63486,#63487,#63488,#63489));
#14280=EDGE_LOOP('',(#63490,#63491,#63492,#63493));
#14281=EDGE_LOOP('',(#63494,#63495,#63496,#63497));
#14282=EDGE_LOOP('',(#63498,#63499,#63500,#63501));
#14283=EDGE_LOOP('',(#63502,#63503,#63504,#63505));
#14284=EDGE_LOOP('',(#63506,#63507,#63508,#63509));
#14285=EDGE_LOOP('',(#63510,#63511,#63512,#63513,#63514,#63515));
#14286=EDGE_LOOP('',(#63516,#63517,#63518,#63519));
#14287=EDGE_LOOP('',(#63520,#63521,#63522,#63523));
#14288=EDGE_LOOP('',(#63524,#63525,#63526,#63527,#63528,#63529));
#14289=EDGE_LOOP('',(#63530,#63531,#63532,#63533));
#14290=EDGE_LOOP('',(#63534,#63535,#63536,#63537));
#14291=EDGE_LOOP('',(#63538,#63539,#63540,#63541));
#14292=EDGE_LOOP('',(#63542,#63543,#63544,#63545));
#14293=EDGE_LOOP('',(#63546,#63547,#63548,#63549));
#14294=EDGE_LOOP('',(#63550,#63551,#63552,#63553,#63554,#63555));
#14295=EDGE_LOOP('',(#63556,#63557,#63558,#63559));
#14296=EDGE_LOOP('',(#63560,#63561,#63562,#63563));
#14297=EDGE_LOOP('',(#63564,#63565,#63566,#63567,#63568,#63569));
#14298=EDGE_LOOP('',(#63570,#63571,#63572,#63573));
#14299=EDGE_LOOP('',(#63574,#63575,#63576,#63577));
#14300=EDGE_LOOP('',(#63578,#63579,#63580,#63581));
#14301=EDGE_LOOP('',(#63582,#63583,#63584,#63585));
#14302=EDGE_LOOP('',(#63586,#63587,#63588,#63589));
#14303=EDGE_LOOP('',(#63590,#63591,#63592,#63593,#63594,#63595));
#14304=EDGE_LOOP('',(#63596,#63597,#63598,#63599));
#14305=EDGE_LOOP('',(#63600,#63601,#63602,#63603));
#14306=EDGE_LOOP('',(#63604,#63605,#63606,#63607,#63608,#63609));
#14307=EDGE_LOOP('',(#63610,#63611,#63612,#63613));
#14308=EDGE_LOOP('',(#63614,#63615,#63616,#63617));
#14309=EDGE_LOOP('',(#63618,#63619,#63620,#63621));
#14310=EDGE_LOOP('',(#63622,#63623,#63624,#63625));
#14311=EDGE_LOOP('',(#63626,#63627,#63628,#63629));
#14312=EDGE_LOOP('',(#63630,#63631,#63632,#63633,#63634,#63635));
#14313=EDGE_LOOP('',(#63636,#63637,#63638,#63639));
#14314=EDGE_LOOP('',(#63640,#63641,#63642,#63643));
#14315=EDGE_LOOP('',(#63644,#63645,#63646,#63647,#63648,#63649));
#14316=EDGE_LOOP('',(#63650,#63651,#63652,#63653));
#14317=EDGE_LOOP('',(#63654,#63655,#63656,#63657));
#14318=EDGE_LOOP('',(#63658,#63659,#63660,#63661));
#14319=EDGE_LOOP('',(#63662,#63663,#63664,#63665));
#14320=EDGE_LOOP('',(#63666,#63667,#63668,#63669));
#14321=EDGE_LOOP('',(#63670,#63671,#63672,#63673,#63674,#63675));
#14322=EDGE_LOOP('',(#63676,#63677,#63678,#63679));
#14323=EDGE_LOOP('',(#63680,#63681,#63682,#63683));
#14324=EDGE_LOOP('',(#63684,#63685,#63686,#63687,#63688,#63689));
#14325=EDGE_LOOP('',(#63690,#63691,#63692,#63693));
#14326=EDGE_LOOP('',(#63694,#63695,#63696,#63697));
#14327=EDGE_LOOP('',(#63698,#63699,#63700,#63701));
#14328=EDGE_LOOP('',(#63702,#63703,#63704,#63705));
#14329=EDGE_LOOP('',(#63706,#63707,#63708,#63709));
#14330=EDGE_LOOP('',(#63710,#63711,#63712,#63713,#63714,#63715));
#14331=EDGE_LOOP('',(#63716,#63717,#63718,#63719));
#14332=EDGE_LOOP('',(#63720,#63721,#63722,#63723));
#14333=EDGE_LOOP('',(#63724,#63725,#63726,#63727,#63728,#63729));
#14334=EDGE_LOOP('',(#63730,#63731,#63732,#63733));
#14335=EDGE_LOOP('',(#63734,#63735,#63736,#63737));
#14336=EDGE_LOOP('',(#63738,#63739,#63740,#63741));
#14337=EDGE_LOOP('',(#63742,#63743,#63744,#63745));
#14338=EDGE_LOOP('',(#63746,#63747,#63748,#63749));
#14339=EDGE_LOOP('',(#63750,#63751,#63752,#63753,#63754,#63755));
#14340=EDGE_LOOP('',(#63756,#63757,#63758,#63759));
#14341=EDGE_LOOP('',(#63760,#63761,#63762,#63763));
#14342=EDGE_LOOP('',(#63764,#63765,#63766,#63767,#63768,#63769));
#14343=EDGE_LOOP('',(#63770,#63771,#63772,#63773));
#14344=EDGE_LOOP('',(#63774,#63775,#63776,#63777));
#14345=EDGE_LOOP('',(#63778,#63779,#63780,#63781));
#14346=EDGE_LOOP('',(#63782,#63783,#63784,#63785));
#14347=EDGE_LOOP('',(#63786,#63787,#63788,#63789));
#14348=EDGE_LOOP('',(#63790,#63791,#63792,#63793,#63794,#63795));
#14349=EDGE_LOOP('',(#63796,#63797,#63798,#63799));
#14350=EDGE_LOOP('',(#63800,#63801,#63802,#63803));
#14351=EDGE_LOOP('',(#63804,#63805,#63806,#63807,#63808,#63809));
#14352=EDGE_LOOP('',(#63810,#63811,#63812,#63813));
#14353=EDGE_LOOP('',(#63814,#63815,#63816,#63817));
#14354=EDGE_LOOP('',(#63818,#63819,#63820,#63821));
#14355=EDGE_LOOP('',(#63822,#63823,#63824,#63825));
#14356=EDGE_LOOP('',(#63826,#63827,#63828,#63829));
#14357=EDGE_LOOP('',(#63830,#63831,#63832,#63833,#63834,#63835));
#14358=EDGE_LOOP('',(#63836,#63837,#63838,#63839));
#14359=EDGE_LOOP('',(#63840,#63841,#63842,#63843));
#14360=EDGE_LOOP('',(#63844,#63845,#63846,#63847,#63848,#63849));
#14361=EDGE_LOOP('',(#63850,#63851,#63852,#63853));
#14362=EDGE_LOOP('',(#63854,#63855,#63856,#63857));
#14363=EDGE_LOOP('',(#63858,#63859,#63860,#63861));
#14364=EDGE_LOOP('',(#63862,#63863,#63864,#63865));
#14365=EDGE_LOOP('',(#63866,#63867,#63868,#63869));
#14366=EDGE_LOOP('',(#63870,#63871,#63872,#63873,#63874,#63875));
#14367=EDGE_LOOP('',(#63876,#63877,#63878,#63879));
#14368=EDGE_LOOP('',(#63880,#63881,#63882,#63883));
#14369=EDGE_LOOP('',(#63884,#63885,#63886,#63887,#63888,#63889));
#14370=EDGE_LOOP('',(#63890,#63891,#63892,#63893));
#14371=EDGE_LOOP('',(#63894,#63895,#63896,#63897));
#14372=EDGE_LOOP('',(#63898,#63899,#63900,#63901));
#14373=EDGE_LOOP('',(#63902,#63903,#63904,#63905));
#14374=EDGE_LOOP('',(#63906,#63907,#63908,#63909));
#14375=EDGE_LOOP('',(#63910,#63911,#63912,#63913,#63914,#63915));
#14376=EDGE_LOOP('',(#63916,#63917,#63918,#63919));
#14377=EDGE_LOOP('',(#63920,#63921,#63922,#63923));
#14378=EDGE_LOOP('',(#63924,#63925,#63926,#63927,#63928,#63929));
#14379=EDGE_LOOP('',(#63930,#63931,#63932,#63933));
#14380=EDGE_LOOP('',(#63934,#63935,#63936,#63937));
#14381=EDGE_LOOP('',(#63938,#63939,#63940,#63941));
#14382=EDGE_LOOP('',(#63942,#63943,#63944,#63945));
#14383=EDGE_LOOP('',(#63946,#63947,#63948,#63949));
#14384=EDGE_LOOP('',(#63950,#63951,#63952,#63953,#63954,#63955));
#14385=EDGE_LOOP('',(#63956,#63957,#63958,#63959));
#14386=EDGE_LOOP('',(#63960,#63961,#63962,#63963));
#14387=EDGE_LOOP('',(#63964,#63965,#63966,#63967,#63968,#63969));
#14388=EDGE_LOOP('',(#63970,#63971,#63972,#63973));
#14389=EDGE_LOOP('',(#63974,#63975,#63976,#63977));
#14390=EDGE_LOOP('',(#63978,#63979,#63980,#63981));
#14391=EDGE_LOOP('',(#63982,#63983,#63984,#63985));
#14392=EDGE_LOOP('',(#63986,#63987,#63988,#63989));
#14393=EDGE_LOOP('',(#63990,#63991,#63992,#63993,#63994,#63995));
#14394=EDGE_LOOP('',(#63996,#63997,#63998,#63999));
#14395=EDGE_LOOP('',(#64000,#64001,#64002,#64003));
#14396=EDGE_LOOP('',(#64004,#64005,#64006,#64007,#64008,#64009));
#14397=EDGE_LOOP('',(#64010,#64011,#64012,#64013));
#14398=EDGE_LOOP('',(#64014,#64015,#64016,#64017));
#14399=EDGE_LOOP('',(#64018,#64019,#64020,#64021));
#14400=EDGE_LOOP('',(#64022,#64023,#64024,#64025));
#14401=EDGE_LOOP('',(#64026,#64027,#64028,#64029));
#14402=EDGE_LOOP('',(#64030,#64031,#64032,#64033,#64034,#64035));
#14403=EDGE_LOOP('',(#64036,#64037,#64038,#64039));
#14404=EDGE_LOOP('',(#64040,#64041,#64042,#64043));
#14405=EDGE_LOOP('',(#64044,#64045,#64046,#64047,#64048,#64049));
#14406=EDGE_LOOP('',(#64050,#64051,#64052,#64053));
#14407=EDGE_LOOP('',(#64054,#64055,#64056,#64057));
#14408=EDGE_LOOP('',(#64058,#64059,#64060,#64061));
#14409=EDGE_LOOP('',(#64062,#64063,#64064,#64065));
#14410=EDGE_LOOP('',(#64066,#64067,#64068,#64069));
#14411=EDGE_LOOP('',(#64070,#64071,#64072,#64073,#64074,#64075));
#14412=EDGE_LOOP('',(#64076,#64077,#64078,#64079));
#14413=EDGE_LOOP('',(#64080,#64081,#64082,#64083));
#14414=EDGE_LOOP('',(#64084,#64085,#64086,#64087,#64088,#64089));
#14415=EDGE_LOOP('',(#64090,#64091,#64092,#64093));
#14416=EDGE_LOOP('',(#64094,#64095,#64096,#64097));
#14417=EDGE_LOOP('',(#64098,#64099,#64100,#64101));
#14418=EDGE_LOOP('',(#64102,#64103,#64104,#64105));
#14419=EDGE_LOOP('',(#64106,#64107,#64108,#64109));
#14420=EDGE_LOOP('',(#64110,#64111,#64112,#64113,#64114,#64115));
#14421=EDGE_LOOP('',(#64116,#64117,#64118,#64119));
#14422=EDGE_LOOP('',(#64120,#64121,#64122,#64123));
#14423=EDGE_LOOP('',(#64124,#64125,#64126,#64127,#64128,#64129));
#14424=EDGE_LOOP('',(#64130,#64131,#64132,#64133));
#14425=EDGE_LOOP('',(#64134,#64135,#64136,#64137));
#14426=EDGE_LOOP('',(#64138,#64139,#64140,#64141));
#14427=EDGE_LOOP('',(#64142,#64143,#64144,#64145));
#14428=EDGE_LOOP('',(#64146,#64147,#64148,#64149));
#14429=EDGE_LOOP('',(#64150,#64151,#64152,#64153,#64154,#64155));
#14430=EDGE_LOOP('',(#64156,#64157,#64158,#64159));
#14431=EDGE_LOOP('',(#64160,#64161,#64162,#64163));
#14432=EDGE_LOOP('',(#64164,#64165,#64166,#64167,#64168,#64169));
#14433=EDGE_LOOP('',(#64170,#64171,#64172,#64173));
#14434=EDGE_LOOP('',(#64174,#64175,#64176,#64177));
#14435=EDGE_LOOP('',(#64178,#64179,#64180,#64181));
#14436=EDGE_LOOP('',(#64182,#64183,#64184,#64185));
#14437=EDGE_LOOP('',(#64186,#64187,#64188,#64189));
#14438=EDGE_LOOP('',(#64190,#64191,#64192,#64193,#64194,#64195));
#14439=EDGE_LOOP('',(#64196,#64197,#64198,#64199));
#14440=EDGE_LOOP('',(#64200,#64201,#64202,#64203));
#14441=EDGE_LOOP('',(#64204,#64205,#64206,#64207,#64208,#64209));
#14442=EDGE_LOOP('',(#64210,#64211,#64212,#64213));
#14443=EDGE_LOOP('',(#64214,#64215,#64216,#64217));
#14444=EDGE_LOOP('',(#64218,#64219,#64220,#64221));
#14445=EDGE_LOOP('',(#64222,#64223,#64224,#64225));
#14446=EDGE_LOOP('',(#64226,#64227,#64228,#64229));
#14447=EDGE_LOOP('',(#64230,#64231,#64232,#64233,#64234,#64235));
#14448=EDGE_LOOP('',(#64236,#64237,#64238,#64239));
#14449=EDGE_LOOP('',(#64240,#64241,#64242,#64243));
#14450=EDGE_LOOP('',(#64244,#64245,#64246,#64247,#64248,#64249));
#14451=EDGE_LOOP('',(#64250,#64251,#64252,#64253));
#14452=EDGE_LOOP('',(#64254,#64255,#64256,#64257));
#14453=EDGE_LOOP('',(#64258,#64259,#64260,#64261));
#14454=EDGE_LOOP('',(#64262,#64263,#64264,#64265));
#14455=EDGE_LOOP('',(#64266,#64267,#64268,#64269));
#14456=EDGE_LOOP('',(#64270,#64271,#64272,#64273,#64274,#64275));
#14457=EDGE_LOOP('',(#64276,#64277,#64278,#64279));
#14458=EDGE_LOOP('',(#64280,#64281,#64282,#64283));
#14459=EDGE_LOOP('',(#64284,#64285,#64286,#64287,#64288,#64289));
#14460=EDGE_LOOP('',(#64290,#64291,#64292,#64293));
#14461=EDGE_LOOP('',(#64294,#64295,#64296,#64297));
#14462=EDGE_LOOP('',(#64298,#64299,#64300,#64301));
#14463=EDGE_LOOP('',(#64302,#64303,#64304,#64305));
#14464=EDGE_LOOP('',(#64306,#64307,#64308,#64309));
#14465=EDGE_LOOP('',(#64310,#64311,#64312,#64313,#64314,#64315));
#14466=EDGE_LOOP('',(#64316,#64317,#64318,#64319));
#14467=EDGE_LOOP('',(#64320,#64321,#64322,#64323));
#14468=EDGE_LOOP('',(#64324,#64325,#64326,#64327,#64328,#64329));
#14469=EDGE_LOOP('',(#64330,#64331,#64332,#64333));
#14470=EDGE_LOOP('',(#64334,#64335,#64336,#64337));
#14471=EDGE_LOOP('',(#64338,#64339,#64340,#64341));
#14472=EDGE_LOOP('',(#64342,#64343,#64344,#64345));
#14473=EDGE_LOOP('',(#64346,#64347,#64348,#64349));
#14474=EDGE_LOOP('',(#64350));
#14475=EDGE_LOOP('',(#64351));
#14476=EDGE_LOOP('',(#64352,#64353,#64354,#64355,#64356,#64357));
#14477=EDGE_LOOP('',(#64358,#64359,#64360,#64361));
#14478=EDGE_LOOP('',(#64362,#64363,#64364,#64365));
#14479=EDGE_LOOP('',(#64366,#64367,#64368,#64369,#64370,#64371));
#14480=EDGE_LOOP('',(#64372,#64373,#64374,#64375));
#14481=EDGE_LOOP('',(#64376));
#14482=EDGE_LOOP('',(#64377));
#14483=EDGE_LOOP('',(#64378));
#14484=EDGE_LOOP('',(#64379));
#14485=EDGE_LOOP('',(#64380,#64381,#64382,#64383));
#14486=EDGE_LOOP('',(#64384,#64385,#64386,#64387));
#14487=EDGE_LOOP('',(#64388,#64389,#64390,#64391));
#14488=EDGE_LOOP('',(#64392,#64393,#64394,#64395));
#14489=EDGE_LOOP('',(#64396,#64397,#64398,#64399));
#14490=EDGE_LOOP('',(#64400,#64401,#64402,#64403,#64404,#64405,#64406,#64407,
#64408,#64409,#64410,#64411));
#14491=EDGE_LOOP('',(#64412,#64413,#64414,#64415,#64416,#64417,#64418,#64419,
#64420,#64421,#64422,#64423));
#14492=EDGE_LOOP('',(#64424,#64425,#64426,#64427));
#14493=EDGE_LOOP('',(#64428,#64429,#64430,#64431));
#14494=EDGE_LOOP('',(#64432,#64433,#64434,#64435));
#14495=EDGE_LOOP('',(#64436,#64437,#64438,#64439));
#14496=EDGE_LOOP('',(#64440,#64441,#64442,#64443,#64444));
#14497=EDGE_LOOP('',(#64445,#64446,#64447,#64448));
#14498=EDGE_LOOP('',(#64449,#64450,#64451,#64452));
#14499=EDGE_LOOP('',(#64453,#64454,#64455,#64456));
#14500=EDGE_LOOP('',(#64457,#64458,#64459,#64460));
#14501=EDGE_LOOP('',(#64461,#64462,#64463,#64464,#64465));
#14502=EDGE_LOOP('',(#64466,#64467,#64468,#64469));
#14503=EDGE_LOOP('',(#64470,#64471,#64472,#64473));
#14504=EDGE_LOOP('',(#64474,#64475,#64476,#64477));
#14505=EDGE_LOOP('',(#64478,#64479,#64480,#64481));
#14506=EDGE_LOOP('',(#64482,#64483,#64484,#64485));
#14507=EDGE_LOOP('',(#64486,#64487,#64488,#64489));
#14508=EDGE_LOOP('',(#64490,#64491,#64492,#64493));
#14509=EDGE_LOOP('',(#64494,#64495,#64496,#64497));
#14510=EDGE_LOOP('',(#64498,#64499,#64500,#64501));
#14511=EDGE_LOOP('',(#64502,#64503,#64504,#64505,#64506));
#14512=EDGE_LOOP('',(#64507,#64508,#64509,#64510,#64511));
#14513=EDGE_LOOP('',(#64512,#64513,#64514,#64515));
#14514=EDGE_LOOP('',(#64516,#64517,#64518,#64519));
#14515=EDGE_LOOP('',(#64520,#64521,#64522,#64523));
#14516=EDGE_LOOP('',(#64524,#64525,#64526,#64527));
#14517=EDGE_LOOP('',(#64528,#64529,#64530,#64531));
#14518=EDGE_LOOP('',(#64532,#64533,#64534,#64535));
#14519=EDGE_LOOP('',(#64536,#64537,#64538,#64539));
#14520=EDGE_LOOP('',(#64540,#64541,#64542,#64543));
#14521=EDGE_LOOP('',(#64544,#64545,#64546,#64547,#64548));
#14522=EDGE_LOOP('',(#64549,#64550,#64551,#64552));
#14523=EDGE_LOOP('',(#64553,#64554,#64555,#64556,#64557,#64558,#64559,#64560,
#64561,#64562,#64563,#64564));
#14524=EDGE_LOOP('',(#64565,#64566,#64567,#64568,#64569,#64570,#64571,#64572,
#64573,#64574,#64575,#64576));
#14525=EDGE_LOOP('',(#64577,#64578,#64579,#64580));
#14526=EDGE_LOOP('',(#64581,#64582,#64583,#64584,#64585,#64586,#64587,#64588,
#64589,#64590,#64591,#64592));
#14527=EDGE_LOOP('',(#64593,#64594,#64595,#64596,#64597,#64598,#64599,#64600,
#64601,#64602,#64603,#64604));
#14528=EDGE_LOOP('',(#64605,#64606,#64607,#64608));
#14529=EDGE_LOOP('',(#64609,#64610,#64611,#64612,#64613,#64614,#64615,#64616,
#64617,#64618,#64619,#64620));
#14530=EDGE_LOOP('',(#64621,#64622,#64623,#64624,#64625,#64626,#64627,#64628,
#64629,#64630,#64631,#64632));
#14531=EDGE_LOOP('',(#64633,#64634,#64635,#64636));
#14532=EDGE_LOOP('',(#64637,#64638,#64639,#64640,#64641,#64642,#64643,#64644,
#64645,#64646,#64647,#64648));
#14533=EDGE_LOOP('',(#64649,#64650,#64651,#64652,#64653,#64654,#64655,#64656,
#64657,#64658,#64659,#64660));
#14534=EDGE_LOOP('',(#64661,#64662,#64663,#64664));
#14535=EDGE_LOOP('',(#64665,#64666,#64667,#64668,#64669,#64670,#64671,#64672,
#64673,#64674,#64675,#64676));
#14536=EDGE_LOOP('',(#64677,#64678,#64679,#64680,#64681,#64682,#64683,#64684,
#64685,#64686,#64687,#64688));
#14537=EDGE_LOOP('',(#64689,#64690,#64691,#64692));
#14538=EDGE_LOOP('',(#64693,#64694,#64695,#64696,#64697,#64698,#64699,#64700,
#64701,#64702,#64703,#64704));
#14539=EDGE_LOOP('',(#64705,#64706,#64707,#64708,#64709,#64710,#64711,#64712,
#64713,#64714,#64715,#64716));
#14540=EDGE_LOOP('',(#64717,#64718,#64719,#64720));
#14541=EDGE_LOOP('',(#64721,#64722,#64723,#64724,#64725,#64726,#64727,#64728,
#64729,#64730,#64731,#64732));
#14542=EDGE_LOOP('',(#64733,#64734,#64735,#64736,#64737,#64738,#64739,#64740,
#64741,#64742,#64743,#64744));
#14543=EDGE_LOOP('',(#64745,#64746,#64747,#64748));
#14544=EDGE_LOOP('',(#64749,#64750,#64751,#64752,#64753,#64754,#64755,#64756,
#64757,#64758,#64759,#64760));
#14545=EDGE_LOOP('',(#64761,#64762,#64763,#64764,#64765,#64766,#64767,#64768,
#64769,#64770,#64771,#64772));
#14546=EDGE_LOOP('',(#64773,#64774,#64775,#64776));
#14547=EDGE_LOOP('',(#64777,#64778,#64779,#64780,#64781,#64782,#64783,#64784,
#64785,#64786,#64787,#64788));
#14548=EDGE_LOOP('',(#64789,#64790,#64791,#64792,#64793,#64794,#64795,#64796,
#64797,#64798,#64799,#64800));
#14549=EDGE_LOOP('',(#64801,#64802,#64803,#64804));
#14550=EDGE_LOOP('',(#64805,#64806,#64807,#64808,#64809,#64810,#64811,#64812,
#64813,#64814,#64815,#64816));
#14551=EDGE_LOOP('',(#64817,#64818,#64819,#64820,#64821,#64822,#64823,#64824,
#64825,#64826,#64827,#64828));
#14552=EDGE_LOOP('',(#64829,#64830,#64831,#64832));
#14553=EDGE_LOOP('',(#64833,#64834,#64835,#64836,#64837,#64838,#64839,#64840,
#64841,#64842,#64843,#64844));
#14554=EDGE_LOOP('',(#64845,#64846,#64847,#64848,#64849,#64850,#64851,#64852,
#64853,#64854,#64855,#64856));
#14555=EDGE_LOOP('',(#64857,#64858,#64859,#64860));
#14556=EDGE_LOOP('',(#64861,#64862,#64863,#64864,#64865,#64866,#64867,#64868,
#64869,#64870,#64871,#64872));
#14557=EDGE_LOOP('',(#64873,#64874,#64875,#64876,#64877,#64878,#64879,#64880,
#64881,#64882,#64883,#64884));
#14558=EDGE_LOOP('',(#64885,#64886,#64887,#64888));
#14559=EDGE_LOOP('',(#64889,#64890,#64891,#64892,#64893,#64894,#64895,#64896,
#64897,#64898,#64899,#64900));
#14560=EDGE_LOOP('',(#64901,#64902,#64903,#64904,#64905,#64906,#64907,#64908,
#64909,#64910,#64911,#64912));
#14561=EDGE_LOOP('',(#64913,#64914,#64915,#64916));
#14562=EDGE_LOOP('',(#64917,#64918,#64919,#64920,#64921,#64922,#64923,#64924,
#64925,#64926,#64927,#64928));
#14563=EDGE_LOOP('',(#64929,#64930,#64931,#64932,#64933,#64934,#64935,#64936,
#64937,#64938,#64939,#64940));
#14564=EDGE_LOOP('',(#64941,#64942,#64943,#64944));
#14565=EDGE_LOOP('',(#64945,#64946,#64947,#64948,#64949,#64950,#64951,#64952,
#64953,#64954,#64955,#64956));
#14566=EDGE_LOOP('',(#64957,#64958,#64959,#64960,#64961,#64962,#64963,#64964,
#64965,#64966,#64967,#64968));
#14567=EDGE_LOOP('',(#64969,#64970,#64971,#64972));
#14568=EDGE_LOOP('',(#64973,#64974,#64975,#64976,#64977,#64978,#64979,#64980,
#64981,#64982,#64983,#64984));
#14569=EDGE_LOOP('',(#64985,#64986,#64987,#64988,#64989,#64990,#64991,#64992,
#64993,#64994,#64995,#64996));
#14570=EDGE_LOOP('',(#64997,#64998,#64999,#65000));
#14571=EDGE_LOOP('',(#65001,#65002,#65003,#65004,#65005,#65006,#65007,#65008,
#65009,#65010,#65011,#65012));
#14572=EDGE_LOOP('',(#65013,#65014,#65015,#65016,#65017,#65018,#65019,#65020,
#65021,#65022,#65023,#65024));
#14573=EDGE_LOOP('',(#65025,#65026,#65027,#65028));
#14574=EDGE_LOOP('',(#65029,#65030,#65031,#65032,#65033,#65034,#65035,#65036,
#65037,#65038,#65039,#65040));
#14575=EDGE_LOOP('',(#65041,#65042,#65043,#65044,#65045,#65046,#65047,#65048,
#65049,#65050,#65051,#65052));
#14576=EDGE_LOOP('',(#65053,#65054,#65055,#65056));
#14577=EDGE_LOOP('',(#65057,#65058,#65059,#65060,#65061,#65062,#65063,#65064,
#65065,#65066,#65067,#65068));
#14578=EDGE_LOOP('',(#65069,#65070,#65071,#65072,#65073,#65074,#65075,#65076,
#65077,#65078,#65079,#65080));
#14579=EDGE_LOOP('',(#65081,#65082,#65083,#65084));
#14580=EDGE_LOOP('',(#65085,#65086,#65087,#65088,#65089,#65090,#65091,#65092,
#65093,#65094,#65095,#65096));
#14581=EDGE_LOOP('',(#65097,#65098,#65099,#65100,#65101,#65102,#65103,#65104,
#65105,#65106,#65107,#65108));
#14582=EDGE_LOOP('',(#65109,#65110,#65111,#65112));
#14583=EDGE_LOOP('',(#65113,#65114,#65115,#65116,#65117,#65118,#65119,#65120,
#65121,#65122,#65123,#65124));
#14584=EDGE_LOOP('',(#65125,#65126,#65127,#65128,#65129,#65130,#65131,#65132,
#65133,#65134,#65135,#65136));
#14585=EDGE_LOOP('',(#65137,#65138,#65139,#65140));
#14586=EDGE_LOOP('',(#65141,#65142,#65143,#65144,#65145,#65146,#65147,#65148,
#65149,#65150,#65151,#65152));
#14587=EDGE_LOOP('',(#65153,#65154,#65155,#65156,#65157,#65158,#65159,#65160,
#65161,#65162,#65163,#65164));
#14588=EDGE_LOOP('',(#65165,#65166,#65167,#65168));
#14589=EDGE_LOOP('',(#65169,#65170,#65171,#65172,#65173,#65174,#65175,#65176,
#65177,#65178,#65179,#65180));
#14590=EDGE_LOOP('',(#65181,#65182,#65183,#65184,#65185,#65186,#65187,#65188,
#65189,#65190,#65191,#65192));
#14591=EDGE_LOOP('',(#65193,#65194,#65195,#65196));
#14592=EDGE_LOOP('',(#65197,#65198,#65199,#65200,#65201,#65202,#65203,#65204,
#65205,#65206,#65207,#65208));
#14593=EDGE_LOOP('',(#65209,#65210,#65211,#65212,#65213,#65214,#65215,#65216,
#65217,#65218,#65219,#65220));
#14594=EDGE_LOOP('',(#65221,#65222,#65223,#65224));
#14595=EDGE_LOOP('',(#65225,#65226,#65227,#65228,#65229,#65230,#65231,#65232,
#65233,#65234,#65235,#65236));
#14596=EDGE_LOOP('',(#65237,#65238,#65239,#65240,#65241,#65242,#65243,#65244,
#65245,#65246,#65247,#65248));
#14597=EDGE_LOOP('',(#65249,#65250,#65251,#65252));
#14598=EDGE_LOOP('',(#65253,#65254,#65255,#65256,#65257,#65258,#65259,#65260,
#65261,#65262,#65263,#65264));
#14599=EDGE_LOOP('',(#65265,#65266,#65267,#65268,#65269,#65270,#65271,#65272,
#65273,#65274,#65275,#65276));
#14600=EDGE_LOOP('',(#65277,#65278,#65279,#65280));
#14601=EDGE_LOOP('',(#65281,#65282,#65283,#65284,#65285,#65286,#65287,#65288,
#65289,#65290,#65291,#65292));
#14602=EDGE_LOOP('',(#65293,#65294,#65295,#65296,#65297,#65298,#65299,#65300,
#65301,#65302,#65303,#65304));
#14603=EDGE_LOOP('',(#65305,#65306,#65307,#65308));
#14604=EDGE_LOOP('',(#65309,#65310,#65311,#65312,#65313,#65314,#65315,#65316,
#65317,#65318,#65319,#65320));
#14605=EDGE_LOOP('',(#65321,#65322,#65323,#65324,#65325,#65326,#65327,#65328,
#65329,#65330,#65331,#65332));
#14606=EDGE_LOOP('',(#65333,#65334,#65335,#65336));
#14607=EDGE_LOOP('',(#65337,#65338,#65339,#65340,#65341,#65342,#65343,#65344,
#65345,#65346,#65347,#65348));
#14608=EDGE_LOOP('',(#65349,#65350,#65351,#65352,#65353,#65354,#65355,#65356,
#65357,#65358,#65359,#65360));
#14609=EDGE_LOOP('',(#65361,#65362,#65363,#65364));
#14610=EDGE_LOOP('',(#65365,#65366,#65367,#65368,#65369,#65370,#65371,#65372,
#65373,#65374,#65375,#65376));
#14611=EDGE_LOOP('',(#65377,#65378,#65379,#65380,#65381,#65382,#65383,#65384,
#65385,#65386,#65387,#65388));
#14612=EDGE_LOOP('',(#65389,#65390,#65391,#65392));
#14613=EDGE_LOOP('',(#65393,#65394,#65395,#65396,#65397,#65398,#65399,#65400,
#65401,#65402,#65403,#65404));
#14614=EDGE_LOOP('',(#65405,#65406,#65407,#65408,#65409,#65410,#65411,#65412,
#65413,#65414,#65415,#65416));
#14615=EDGE_LOOP('',(#65417,#65418,#65419,#65420));
#14616=EDGE_LOOP('',(#65421,#65422,#65423,#65424,#65425,#65426,#65427,#65428,
#65429,#65430,#65431,#65432));
#14617=EDGE_LOOP('',(#65433,#65434,#65435,#65436,#65437,#65438,#65439,#65440,
#65441,#65442,#65443,#65444));
#14618=EDGE_LOOP('',(#65445,#65446,#65447,#65448));
#14619=EDGE_LOOP('',(#65449,#65450,#65451,#65452,#65453,#65454,#65455,#65456,
#65457,#65458,#65459,#65460));
#14620=EDGE_LOOP('',(#65461,#65462,#65463,#65464,#65465,#65466,#65467,#65468,
#65469,#65470,#65471,#65472));
#14621=EDGE_LOOP('',(#65473,#65474,#65475,#65476));
#14622=EDGE_LOOP('',(#65477,#65478,#65479,#65480,#65481,#65482,#65483,#65484,
#65485,#65486,#65487,#65488));
#14623=EDGE_LOOP('',(#65489,#65490,#65491,#65492,#65493,#65494,#65495,#65496,
#65497,#65498,#65499,#65500));
#14624=EDGE_LOOP('',(#65501,#65502,#65503,#65504));
#14625=EDGE_LOOP('',(#65505,#65506,#65507,#65508,#65509,#65510,#65511,#65512,
#65513,#65514,#65515,#65516));
#14626=EDGE_LOOP('',(#65517,#65518,#65519,#65520,#65521,#65522,#65523,#65524,
#65525,#65526,#65527,#65528));
#14627=EDGE_LOOP('',(#65529,#65530,#65531,#65532));
#14628=EDGE_LOOP('',(#65533,#65534,#65535,#65536,#65537,#65538,#65539,#65540,
#65541,#65542,#65543,#65544));
#14629=EDGE_LOOP('',(#65545,#65546,#65547,#65548,#65549,#65550,#65551,#65552,
#65553,#65554,#65555,#65556));
#14630=EDGE_LOOP('',(#65557,#65558,#65559,#65560));
#14631=EDGE_LOOP('',(#65561,#65562,#65563,#65564,#65565,#65566,#65567,#65568,
#65569,#65570,#65571,#65572));
#14632=EDGE_LOOP('',(#65573,#65574,#65575,#65576,#65577,#65578,#65579,#65580,
#65581,#65582,#65583,#65584));
#14633=EDGE_LOOP('',(#65585,#65586,#65587,#65588));
#14634=EDGE_LOOP('',(#65589,#65590,#65591,#65592,#65593,#65594,#65595,#65596,
#65597,#65598,#65599,#65600));
#14635=EDGE_LOOP('',(#65601,#65602,#65603,#65604,#65605,#65606,#65607,#65608,
#65609,#65610,#65611,#65612));
#14636=EDGE_LOOP('',(#65613,#65614,#65615,#65616));
#14637=EDGE_LOOP('',(#65617,#65618,#65619,#65620,#65621,#65622,#65623,#65624,
#65625,#65626,#65627,#65628));
#14638=EDGE_LOOP('',(#65629,#65630,#65631,#65632,#65633,#65634,#65635,#65636,
#65637,#65638,#65639,#65640));
#14639=EDGE_LOOP('',(#65641,#65642,#65643,#65644));
#14640=EDGE_LOOP('',(#65645,#65646,#65647,#65648,#65649,#65650,#65651,#65652,
#65653,#65654,#65655,#65656));
#14641=EDGE_LOOP('',(#65657,#65658,#65659,#65660,#65661,#65662,#65663,#65664,
#65665,#65666,#65667,#65668));
#14642=EDGE_LOOP('',(#65669,#65670,#65671,#65672));
#14643=EDGE_LOOP('',(#65673,#65674,#65675,#65676,#65677,#65678,#65679,#65680,
#65681,#65682,#65683,#65684));
#14644=EDGE_LOOP('',(#65685,#65686,#65687,#65688,#65689,#65690,#65691,#65692,
#65693,#65694,#65695,#65696));
#14645=EDGE_LOOP('',(#65697,#65698,#65699,#65700));
#14646=EDGE_LOOP('',(#65701,#65702,#65703,#65704,#65705,#65706,#65707,#65708,
#65709,#65710,#65711,#65712));
#14647=EDGE_LOOP('',(#65713,#65714,#65715,#65716,#65717,#65718,#65719,#65720,
#65721,#65722,#65723,#65724));
#14648=EDGE_LOOP('',(#65725,#65726,#65727,#65728));
#14649=EDGE_LOOP('',(#65729,#65730,#65731,#65732,#65733,#65734,#65735,#65736,
#65737,#65738,#65739,#65740));
#14650=EDGE_LOOP('',(#65741,#65742,#65743,#65744,#65745,#65746,#65747,#65748,
#65749,#65750,#65751,#65752));
#14651=EDGE_LOOP('',(#65753,#65754,#65755,#65756));
#14652=EDGE_LOOP('',(#65757,#65758,#65759,#65760,#65761,#65762,#65763,#65764,
#65765,#65766,#65767,#65768));
#14653=EDGE_LOOP('',(#65769,#65770,#65771,#65772,#65773,#65774,#65775,#65776,
#65777,#65778,#65779,#65780));
#14654=EDGE_LOOP('',(#65781,#65782,#65783,#65784));
#14655=EDGE_LOOP('',(#65785,#65786,#65787,#65788,#65789,#65790,#65791,#65792,
#65793,#65794,#65795,#65796));
#14656=EDGE_LOOP('',(#65797,#65798,#65799,#65800,#65801,#65802,#65803,#65804,
#65805,#65806,#65807,#65808));
#14657=EDGE_LOOP('',(#65809,#65810,#65811,#65812));
#14658=EDGE_LOOP('',(#65813,#65814,#65815,#65816,#65817,#65818,#65819,#65820,
#65821,#65822,#65823,#65824));
#14659=EDGE_LOOP('',(#65825,#65826,#65827,#65828,#65829,#65830,#65831,#65832,
#65833,#65834,#65835,#65836));
#14660=EDGE_LOOP('',(#65837,#65838,#65839,#65840));
#14661=EDGE_LOOP('',(#65841,#65842,#65843,#65844,#65845,#65846,#65847,#65848,
#65849,#65850,#65851,#65852));
#14662=EDGE_LOOP('',(#65853,#65854,#65855,#65856,#65857,#65858,#65859,#65860,
#65861,#65862,#65863,#65864));
#14663=EDGE_LOOP('',(#65865,#65866,#65867,#65868));
#14664=EDGE_LOOP('',(#65869,#65870,#65871,#65872,#65873,#65874,#65875,#65876,
#65877,#65878,#65879,#65880));
#14665=EDGE_LOOP('',(#65881,#65882,#65883,#65884,#65885,#65886,#65887,#65888,
#65889,#65890,#65891,#65892));
#14666=EDGE_LOOP('',(#65893,#65894,#65895,#65896));
#14667=EDGE_LOOP('',(#65897,#65898,#65899,#65900,#65901,#65902,#65903,#65904,
#65905,#65906,#65907,#65908));
#14668=EDGE_LOOP('',(#65909,#65910,#65911,#65912,#65913,#65914,#65915,#65916,
#65917,#65918,#65919,#65920));
#14669=EDGE_LOOP('',(#65921,#65922,#65923,#65924));
#14670=EDGE_LOOP('',(#65925,#65926,#65927,#65928,#65929,#65930,#65931,#65932,
#65933,#65934,#65935,#65936));
#14671=EDGE_LOOP('',(#65937,#65938,#65939,#65940,#65941,#65942,#65943,#65944,
#65945,#65946,#65947,#65948));
#14672=EDGE_LOOP('',(#65949,#65950,#65951,#65952));
#14673=EDGE_LOOP('',(#65953,#65954,#65955,#65956,#65957,#65958,#65959,#65960,
#65961,#65962,#65963,#65964));
#14674=EDGE_LOOP('',(#65965,#65966,#65967,#65968,#65969,#65970,#65971,#65972,
#65973,#65974,#65975,#65976));
#14675=EDGE_LOOP('',(#65977,#65978,#65979,#65980));
#14676=EDGE_LOOP('',(#65981,#65982,#65983,#65984,#65985,#65986,#65987,#65988,
#65989,#65990,#65991,#65992));
#14677=EDGE_LOOP('',(#65993,#65994,#65995,#65996,#65997,#65998,#65999,#66000,
#66001,#66002,#66003,#66004));
#14678=EDGE_LOOP('',(#66005,#66006,#66007,#66008));
#14679=EDGE_LOOP('',(#66009,#66010,#66011,#66012,#66013,#66014,#66015,#66016,
#66017,#66018,#66019,#66020));
#14680=EDGE_LOOP('',(#66021,#66022,#66023,#66024,#66025,#66026,#66027,#66028,
#66029,#66030,#66031,#66032));
#14681=EDGE_LOOP('',(#66033,#66034,#66035,#66036));
#14682=EDGE_LOOP('',(#66037,#66038,#66039,#66040,#66041,#66042,#66043,#66044,
#66045,#66046,#66047,#66048));
#14683=EDGE_LOOP('',(#66049,#66050,#66051,#66052,#66053,#66054,#66055,#66056,
#66057,#66058,#66059,#66060));
#14684=EDGE_LOOP('',(#66061,#66062,#66063,#66064));
#14685=EDGE_LOOP('',(#66065,#66066,#66067,#66068,#66069,#66070,#66071,#66072,
#66073,#66074,#66075,#66076));
#14686=EDGE_LOOP('',(#66077,#66078,#66079,#66080,#66081,#66082,#66083,#66084,
#66085,#66086,#66087,#66088));
#14687=EDGE_LOOP('',(#66089,#66090,#66091,#66092));
#14688=EDGE_LOOP('',(#66093,#66094,#66095,#66096,#66097,#66098,#66099,#66100,
#66101,#66102,#66103,#66104));
#14689=EDGE_LOOP('',(#66105,#66106,#66107,#66108,#66109,#66110,#66111,#66112,
#66113,#66114,#66115,#66116));
#14690=EDGE_LOOP('',(#66117,#66118,#66119,#66120));
#14691=EDGE_LOOP('',(#66121,#66122,#66123,#66124,#66125,#66126,#66127,#66128,
#66129,#66130,#66131,#66132));
#14692=EDGE_LOOP('',(#66133,#66134,#66135,#66136,#66137,#66138,#66139,#66140,
#66141,#66142,#66143,#66144));
#14693=EDGE_LOOP('',(#66145,#66146,#66147,#66148));
#14694=EDGE_LOOP('',(#66149,#66150,#66151,#66152,#66153,#66154,#66155,#66156,
#66157,#66158,#66159,#66160));
#14695=EDGE_LOOP('',(#66161,#66162,#66163,#66164,#66165,#66166,#66167,#66168,
#66169,#66170,#66171,#66172));
#14696=EDGE_LOOP('',(#66173,#66174,#66175,#66176));
#14697=EDGE_LOOP('',(#66177,#66178,#66179,#66180,#66181,#66182,#66183,#66184,
#66185,#66186,#66187,#66188));
#14698=EDGE_LOOP('',(#66189,#66190,#66191,#66192,#66193,#66194,#66195,#66196,
#66197,#66198,#66199,#66200));
#14699=EDGE_LOOP('',(#66201,#66202,#66203,#66204));
#14700=EDGE_LOOP('',(#66205,#66206,#66207,#66208));
#14701=EDGE_LOOP('',(#66209,#66210,#66211,#66212));
#14702=EDGE_LOOP('',(#66213,#66214,#66215,#66216));
#14703=EDGE_LOOP('',(#66217,#66218,#66219,#66220));
#14704=EDGE_LOOP('',(#66221,#66222,#66223,#66224));
#14705=EDGE_LOOP('',(#66225,#66226,#66227,#66228));
#14706=EDGE_LOOP('',(#66229,#66230,#66231,#66232));
#14707=EDGE_LOOP('',(#66233,#66234,#66235,#66236));
#14708=EDGE_LOOP('',(#66237,#66238,#66239,#66240));
#14709=EDGE_LOOP('',(#66241,#66242,#66243,#66244));
#14710=EDGE_LOOP('',(#66245,#66246,#66247,#66248));
#14711=EDGE_LOOP('',(#66249,#66250,#66251,#66252));
#14712=EDGE_LOOP('',(#66253,#66254,#66255,#66256));
#14713=EDGE_LOOP('',(#66257,#66258,#66259,#66260));
#14714=EDGE_LOOP('',(#66261,#66262,#66263,#66264));
#14715=EDGE_LOOP('',(#66265,#66266,#66267,#66268));
#14716=EDGE_LOOP('',(#66269,#66270,#66271,#66272));
#14717=EDGE_LOOP('',(#66273,#66274,#66275,#66276));
#14718=EDGE_LOOP('',(#66277,#66278,#66279,#66280));
#14719=EDGE_LOOP('',(#66281,#66282,#66283,#66284));
#14720=EDGE_LOOP('',(#66285,#66286,#66287,#66288));
#14721=EDGE_LOOP('',(#66289,#66290,#66291,#66292));
#14722=EDGE_LOOP('',(#66293,#66294,#66295,#66296));
#14723=EDGE_LOOP('',(#66297,#66298,#66299,#66300));
#14724=EDGE_LOOP('',(#66301,#66302,#66303,#66304));
#14725=EDGE_LOOP('',(#66305,#66306,#66307,#66308));
#14726=EDGE_LOOP('',(#66309,#66310,#66311,#66312));
#14727=EDGE_LOOP('',(#66313,#66314,#66315,#66316));
#14728=EDGE_LOOP('',(#66317,#66318,#66319,#66320));
#14729=EDGE_LOOP('',(#66321,#66322,#66323,#66324));
#14730=EDGE_LOOP('',(#66325,#66326,#66327,#66328));
#14731=EDGE_LOOP('',(#66329,#66330,#66331,#66332));
#14732=EDGE_LOOP('',(#66333,#66334,#66335,#66336));
#14733=EDGE_LOOP('',(#66337,#66338,#66339,#66340));
#14734=EDGE_LOOP('',(#66341,#66342,#66343,#66344));
#14735=EDGE_LOOP('',(#66345,#66346,#66347,#66348));
#14736=EDGE_LOOP('',(#66349,#66350,#66351,#66352));
#14737=EDGE_LOOP('',(#66353,#66354,#66355,#66356));
#14738=EDGE_LOOP('',(#66357,#66358,#66359,#66360));
#14739=EDGE_LOOP('',(#66361,#66362,#66363,#66364));
#14740=EDGE_LOOP('',(#66365,#66366,#66367,#66368));
#14741=EDGE_LOOP('',(#66369,#66370,#66371,#66372));
#14742=EDGE_LOOP('',(#66373,#66374,#66375,#66376));
#14743=EDGE_LOOP('',(#66377,#66378,#66379,#66380));
#14744=EDGE_LOOP('',(#66381,#66382,#66383,#66384));
#14745=EDGE_LOOP('',(#66385,#66386,#66387,#66388));
#14746=EDGE_LOOP('',(#66389,#66390,#66391,#66392));
#14747=EDGE_LOOP('',(#66393,#66394,#66395,#66396));
#14748=EDGE_LOOP('',(#66397,#66398,#66399,#66400));
#14749=EDGE_LOOP('',(#66401,#66402,#66403,#66404));
#14750=EDGE_LOOP('',(#66405,#66406,#66407,#66408));
#14751=EDGE_LOOP('',(#66409,#66410,#66411,#66412));
#14752=EDGE_LOOP('',(#66413,#66414,#66415,#66416));
#14753=EDGE_LOOP('',(#66417,#66418,#66419,#66420));
#14754=EDGE_LOOP('',(#66421,#66422,#66423,#66424));
#14755=EDGE_LOOP('',(#66425,#66426,#66427,#66428));
#14756=EDGE_LOOP('',(#66429,#66430,#66431,#66432));
#14757=EDGE_LOOP('',(#66433,#66434,#66435,#66436));
#14758=EDGE_LOOP('',(#66437,#66438,#66439,#66440));
#14759=EDGE_LOOP('',(#66441,#66442,#66443,#66444));
#14760=EDGE_LOOP('',(#66445,#66446,#66447,#66448));
#14761=EDGE_LOOP('',(#66449,#66450,#66451,#66452));
#14762=EDGE_LOOP('',(#66453,#66454,#66455,#66456));
#14763=EDGE_LOOP('',(#66457,#66458,#66459,#66460));
#14764=EDGE_LOOP('',(#66461,#66462,#66463,#66464));
#14765=EDGE_LOOP('',(#66465,#66466,#66467,#66468));
#14766=EDGE_LOOP('',(#66469,#66470,#66471,#66472));
#14767=EDGE_LOOP('',(#66473,#66474,#66475,#66476));
#14768=EDGE_LOOP('',(#66477,#66478,#66479,#66480));
#14769=EDGE_LOOP('',(#66481,#66482,#66483,#66484));
#14770=EDGE_LOOP('',(#66485,#66486,#66487,#66488));
#14771=EDGE_LOOP('',(#66489,#66490,#66491,#66492));
#14772=EDGE_LOOP('',(#66493,#66494,#66495,#66496));
#14773=EDGE_LOOP('',(#66497,#66498,#66499,#66500));
#14774=EDGE_LOOP('',(#66501,#66502,#66503,#66504));
#14775=EDGE_LOOP('',(#66505,#66506,#66507,#66508));
#14776=EDGE_LOOP('',(#66509,#66510,#66511,#66512));
#14777=EDGE_LOOP('',(#66513,#66514,#66515,#66516));
#14778=EDGE_LOOP('',(#66517,#66518,#66519,#66520));
#14779=EDGE_LOOP('',(#66521,#66522,#66523,#66524));
#14780=EDGE_LOOP('',(#66525,#66526,#66527,#66528));
#14781=EDGE_LOOP('',(#66529,#66530,#66531,#66532));
#14782=EDGE_LOOP('',(#66533,#66534,#66535,#66536));
#14783=EDGE_LOOP('',(#66537,#66538,#66539,#66540));
#14784=EDGE_LOOP('',(#66541,#66542,#66543,#66544));
#14785=EDGE_LOOP('',(#66545,#66546,#66547,#66548));
#14786=EDGE_LOOP('',(#66549,#66550,#66551,#66552));
#14787=EDGE_LOOP('',(#66553,#66554,#66555,#66556));
#14788=EDGE_LOOP('',(#66557,#66558,#66559,#66560));
#14789=EDGE_LOOP('',(#66561,#66562,#66563,#66564));
#14790=EDGE_LOOP('',(#66565,#66566,#66567,#66568));
#14791=EDGE_LOOP('',(#66569,#66570,#66571,#66572));
#14792=EDGE_LOOP('',(#66573,#66574,#66575,#66576));
#14793=EDGE_LOOP('',(#66577,#66578,#66579,#66580));
#14794=EDGE_LOOP('',(#66581,#66582,#66583,#66584));
#14795=EDGE_LOOP('',(#66585,#66586,#66587,#66588));
#14796=EDGE_LOOP('',(#66589,#66590,#66591,#66592));
#14797=EDGE_LOOP('',(#66593,#66594,#66595,#66596));
#14798=EDGE_LOOP('',(#66597,#66598,#66599,#66600));
#14799=EDGE_LOOP('',(#66601,#66602,#66603,#66604));
#14800=EDGE_LOOP('',(#66605,#66606,#66607,#66608));
#14801=EDGE_LOOP('',(#66609,#66610,#66611,#66612));
#14802=EDGE_LOOP('',(#66613,#66614,#66615,#66616));
#14803=EDGE_LOOP('',(#66617,#66618,#66619,#66620));
#14804=EDGE_LOOP('',(#66621,#66622,#66623,#66624));
#14805=EDGE_LOOP('',(#66625,#66626,#66627,#66628));
#14806=EDGE_LOOP('',(#66629,#66630,#66631,#66632));
#14807=EDGE_LOOP('',(#66633,#66634,#66635,#66636));
#14808=EDGE_LOOP('',(#66637,#66638,#66639,#66640));
#14809=EDGE_LOOP('',(#66641,#66642,#66643,#66644));
#14810=EDGE_LOOP('',(#66645,#66646,#66647,#66648));
#14811=EDGE_LOOP('',(#66649,#66650,#66651,#66652));
#14812=EDGE_LOOP('',(#66653,#66654,#66655,#66656));
#14813=EDGE_LOOP('',(#66657,#66658,#66659,#66660));
#14814=EDGE_LOOP('',(#66661,#66662,#66663,#66664));
#14815=EDGE_LOOP('',(#66665,#66666,#66667,#66668));
#14816=EDGE_LOOP('',(#66669,#66670,#66671,#66672));
#14817=EDGE_LOOP('',(#66673,#66674,#66675,#66676));
#14818=EDGE_LOOP('',(#66677,#66678,#66679,#66680));
#14819=EDGE_LOOP('',(#66681,#66682,#66683,#66684,#66685));
#14820=EDGE_LOOP('',(#66686,#66687,#66688,#66689));
#14821=EDGE_LOOP('',(#66690,#66691,#66692,#66693));
#14822=EDGE_LOOP('',(#66694,#66695,#66696,#66697));
#14823=EDGE_LOOP('',(#66698,#66699,#66700,#66701));
#14824=EDGE_LOOP('',(#66702,#66703,#66704,#66705,#66706));
#14825=EDGE_LOOP('',(#66707,#66708,#66709,#66710));
#14826=EDGE_LOOP('',(#66711,#66712,#66713,#66714));
#14827=EDGE_LOOP('',(#66715,#66716,#66717,#66718));
#14828=EDGE_LOOP('',(#66719,#66720,#66721,#66722));
#14829=EDGE_LOOP('',(#66723,#66724,#66725,#66726));
#14830=EDGE_LOOP('',(#66727,#66728,#66729,#66730));
#14831=EDGE_LOOP('',(#66731,#66732,#66733,#66734));
#14832=EDGE_LOOP('',(#66735,#66736,#66737,#66738));
#14833=EDGE_LOOP('',(#66739,#66740,#66741,#66742));
#14834=EDGE_LOOP('',(#66743,#66744,#66745,#66746));
#14835=EDGE_LOOP('',(#66747,#66748,#66749,#66750,#66751));
#14836=EDGE_LOOP('',(#66752,#66753,#66754,#66755));
#14837=EDGE_LOOP('',(#66756,#66757,#66758,#66759));
#14838=EDGE_LOOP('',(#66760,#66761,#66762,#66763));
#14839=EDGE_LOOP('',(#66764,#66765,#66766,#66767));
#14840=EDGE_LOOP('',(#66768,#66769,#66770,#66771));
#14841=EDGE_LOOP('',(#66772,#66773,#66774,#66775));
#14842=EDGE_LOOP('',(#66776,#66777,#66778,#66779));
#14843=EDGE_LOOP('',(#66780,#66781,#66782,#66783));
#14844=EDGE_LOOP('',(#66784,#66785,#66786,#66787,#66788));
#14845=EDGE_LOOP('',(#66789,#66790,#66791,#66792));
#14846=EDGE_LOOP('',(#66793,#66794,#66795,#66796));
#14847=EDGE_LOOP('',(#66797,#66798,#66799,#66800,#66801));
#14848=EDGE_LOOP('',(#66802,#66803,#66804,#66805));
#14849=EDGE_LOOP('',(#66806,#66807,#66808,#66809));
#14850=EDGE_LOOP('',(#66810,#66811,#66812,#66813));
#14851=EDGE_LOOP('',(#66814,#66815,#66816,#66817));
#14852=EDGE_LOOP('',(#66818,#66819,#66820,#66821,#66822));
#14853=EDGE_LOOP('',(#66823,#66824,#66825,#66826));
#14854=EDGE_LOOP('',(#66827,#66828,#66829,#66830));
#14855=EDGE_LOOP('',(#66831,#66832,#66833,#66834));
#14856=EDGE_LOOP('',(#66835,#66836,#66837,#66838));
#14857=EDGE_LOOP('',(#66839,#66840,#66841,#66842));
#14858=EDGE_LOOP('',(#66843,#66844,#66845,#66846));
#14859=EDGE_LOOP('',(#66847,#66848,#66849,#66850));
#14860=EDGE_LOOP('',(#66851,#66852,#66853,#66854));
#14861=EDGE_LOOP('',(#66855,#66856,#66857,#66858));
#14862=EDGE_LOOP('',(#66859,#66860,#66861,#66862));
#14863=EDGE_LOOP('',(#66863,#66864,#66865,#66866,#66867));
#14864=EDGE_LOOP('',(#66868,#66869,#66870,#66871));
#14865=EDGE_LOOP('',(#66872,#66873,#66874,#66875));
#14866=EDGE_LOOP('',(#66876,#66877,#66878,#66879));
#14867=EDGE_LOOP('',(#66880,#66881,#66882,#66883));
#14868=EDGE_LOOP('',(#66884,#66885,#66886,#66887));
#14869=EDGE_LOOP('',(#66888,#66889,#66890,#66891));
#14870=EDGE_LOOP('',(#66892,#66893,#66894,#66895));
#14871=EDGE_LOOP('',(#66896,#66897,#66898,#66899));
#14872=EDGE_LOOP('',(#66900,#66901,#66902,#66903,#66904));
#14873=EDGE_LOOP('',(#66905,#66906,#66907,#66908));
#14874=EDGE_LOOP('',(#66909,#66910,#66911,#66912));
#14875=EDGE_LOOP('',(#66913,#66914,#66915,#66916,#66917));
#14876=EDGE_LOOP('',(#66918,#66919,#66920,#66921));
#14877=EDGE_LOOP('',(#66922,#66923,#66924,#66925));
#14878=EDGE_LOOP('',(#66926,#66927,#66928,#66929));
#14879=EDGE_LOOP('',(#66930,#66931,#66932,#66933));
#14880=EDGE_LOOP('',(#66934,#66935,#66936,#66937,#66938));
#14881=EDGE_LOOP('',(#66939,#66940,#66941,#66942));
#14882=EDGE_LOOP('',(#66943,#66944,#66945,#66946));
#14883=EDGE_LOOP('',(#66947,#66948,#66949,#66950));
#14884=EDGE_LOOP('',(#66951,#66952,#66953,#66954));
#14885=EDGE_LOOP('',(#66955,#66956,#66957,#66958));
#14886=EDGE_LOOP('',(#66959,#66960,#66961,#66962));
#14887=EDGE_LOOP('',(#66963,#66964,#66965,#66966));
#14888=EDGE_LOOP('',(#66967,#66968,#66969,#66970));
#14889=EDGE_LOOP('',(#66971,#66972,#66973,#66974));
#14890=EDGE_LOOP('',(#66975,#66976,#66977,#66978));
#14891=EDGE_LOOP('',(#66979,#66980,#66981,#66982,#66983));
#14892=EDGE_LOOP('',(#66984,#66985,#66986,#66987));
#14893=EDGE_LOOP('',(#66988,#66989,#66990,#66991));
#14894=EDGE_LOOP('',(#66992,#66993,#66994,#66995));
#14895=EDGE_LOOP('',(#66996,#66997,#66998,#66999));
#14896=EDGE_LOOP('',(#67000,#67001,#67002,#67003));
#14897=EDGE_LOOP('',(#67004,#67005,#67006,#67007));
#14898=EDGE_LOOP('',(#67008,#67009,#67010,#67011));
#14899=EDGE_LOOP('',(#67012,#67013,#67014,#67015));
#14900=EDGE_LOOP('',(#67016,#67017,#67018,#67019,#67020));
#14901=EDGE_LOOP('',(#67021,#67022,#67023,#67024));
#14902=EDGE_LOOP('',(#67025,#67026,#67027,#67028));
#14903=EDGE_LOOP('',(#67029,#67030,#67031,#67032,#67033));
#14904=EDGE_LOOP('',(#67034,#67035,#67036,#67037));
#14905=EDGE_LOOP('',(#67038,#67039,#67040,#67041));
#14906=EDGE_LOOP('',(#67042,#67043,#67044,#67045));
#14907=EDGE_LOOP('',(#67046,#67047,#67048,#67049));
#14908=EDGE_LOOP('',(#67050,#67051,#67052,#67053,#67054));
#14909=EDGE_LOOP('',(#67055,#67056,#67057,#67058));
#14910=EDGE_LOOP('',(#67059,#67060,#67061,#67062));
#14911=EDGE_LOOP('',(#67063,#67064,#67065,#67066));
#14912=EDGE_LOOP('',(#67067,#67068,#67069,#67070));
#14913=EDGE_LOOP('',(#67071,#67072,#67073,#67074));
#14914=EDGE_LOOP('',(#67075,#67076,#67077,#67078));
#14915=EDGE_LOOP('',(#67079,#67080,#67081,#67082));
#14916=EDGE_LOOP('',(#67083,#67084,#67085,#67086));
#14917=EDGE_LOOP('',(#67087,#67088,#67089,#67090));
#14918=EDGE_LOOP('',(#67091,#67092,#67093,#67094));
#14919=EDGE_LOOP('',(#67095,#67096,#67097,#67098,#67099));
#14920=EDGE_LOOP('',(#67100,#67101,#67102,#67103));
#14921=EDGE_LOOP('',(#67104,#67105,#67106,#67107));
#14922=EDGE_LOOP('',(#67108,#67109,#67110,#67111));
#14923=EDGE_LOOP('',(#67112,#67113,#67114,#67115));
#14924=EDGE_LOOP('',(#67116,#67117,#67118,#67119));
#14925=EDGE_LOOP('',(#67120,#67121,#67122,#67123));
#14926=EDGE_LOOP('',(#67124,#67125,#67126,#67127));
#14927=EDGE_LOOP('',(#67128,#67129,#67130,#67131));
#14928=EDGE_LOOP('',(#67132,#67133,#67134,#67135,#67136));
#14929=EDGE_LOOP('',(#67137,#67138,#67139,#67140));
#14930=EDGE_LOOP('',(#67141,#67142,#67143,#67144));
#14931=EDGE_LOOP('',(#67145,#67146,#67147,#67148,#67149));
#14932=EDGE_LOOP('',(#67150,#67151,#67152,#67153));
#14933=EDGE_LOOP('',(#67154,#67155,#67156,#67157));
#14934=EDGE_LOOP('',(#67158,#67159,#67160,#67161));
#14935=EDGE_LOOP('',(#67162,#67163,#67164,#67165));
#14936=EDGE_LOOP('',(#67166,#67167,#67168,#67169,#67170));
#14937=EDGE_LOOP('',(#67171,#67172,#67173,#67174));
#14938=EDGE_LOOP('',(#67175,#67176,#67177,#67178));
#14939=EDGE_LOOP('',(#67179,#67180,#67181,#67182));
#14940=EDGE_LOOP('',(#67183,#67184,#67185,#67186));
#14941=EDGE_LOOP('',(#67187,#67188,#67189,#67190));
#14942=EDGE_LOOP('',(#67191,#67192,#67193,#67194));
#14943=EDGE_LOOP('',(#67195,#67196,#67197,#67198));
#14944=EDGE_LOOP('',(#67199,#67200,#67201,#67202));
#14945=EDGE_LOOP('',(#67203,#67204,#67205,#67206));
#14946=EDGE_LOOP('',(#67207,#67208,#67209,#67210));
#14947=EDGE_LOOP('',(#67211,#67212,#67213,#67214,#67215));
#14948=EDGE_LOOP('',(#67216,#67217,#67218,#67219));
#14949=EDGE_LOOP('',(#67220,#67221,#67222,#67223));
#14950=EDGE_LOOP('',(#67224,#67225,#67226,#67227));
#14951=EDGE_LOOP('',(#67228,#67229,#67230,#67231));
#14952=EDGE_LOOP('',(#67232,#67233,#67234,#67235));
#14953=EDGE_LOOP('',(#67236,#67237,#67238,#67239));
#14954=EDGE_LOOP('',(#67240,#67241,#67242,#67243));
#14955=EDGE_LOOP('',(#67244,#67245,#67246,#67247));
#14956=EDGE_LOOP('',(#67248,#67249,#67250,#67251,#67252));
#14957=EDGE_LOOP('',(#67253,#67254,#67255,#67256));
#14958=EDGE_LOOP('',(#67257,#67258,#67259,#67260));
#14959=EDGE_LOOP('',(#67261,#67262,#67263,#67264,#67265));
#14960=EDGE_LOOP('',(#67266,#67267,#67268,#67269));
#14961=EDGE_LOOP('',(#67270,#67271,#67272,#67273));
#14962=EDGE_LOOP('',(#67274,#67275,#67276,#67277));
#14963=EDGE_LOOP('',(#67278,#67279,#67280,#67281));
#14964=EDGE_LOOP('',(#67282,#67283,#67284,#67285,#67286));
#14965=EDGE_LOOP('',(#67287,#67288,#67289,#67290));
#14966=EDGE_LOOP('',(#67291,#67292,#67293,#67294));
#14967=EDGE_LOOP('',(#67295,#67296,#67297,#67298));
#14968=EDGE_LOOP('',(#67299,#67300,#67301,#67302));
#14969=EDGE_LOOP('',(#67303,#67304,#67305,#67306));
#14970=EDGE_LOOP('',(#67307,#67308,#67309,#67310));
#14971=EDGE_LOOP('',(#67311,#67312,#67313,#67314));
#14972=EDGE_LOOP('',(#67315,#67316,#67317,#67318));
#14973=EDGE_LOOP('',(#67319,#67320,#67321,#67322));
#14974=EDGE_LOOP('',(#67323,#67324,#67325,#67326));
#14975=EDGE_LOOP('',(#67327,#67328,#67329,#67330,#67331));
#14976=EDGE_LOOP('',(#67332,#67333,#67334,#67335));
#14977=EDGE_LOOP('',(#67336,#67337,#67338,#67339));
#14978=EDGE_LOOP('',(#67340,#67341,#67342,#67343));
#14979=EDGE_LOOP('',(#67344,#67345,#67346,#67347));
#14980=EDGE_LOOP('',(#67348,#67349,#67350,#67351));
#14981=EDGE_LOOP('',(#67352,#67353,#67354,#67355));
#14982=EDGE_LOOP('',(#67356,#67357,#67358,#67359));
#14983=EDGE_LOOP('',(#67360,#67361,#67362,#67363));
#14984=EDGE_LOOP('',(#67364,#67365,#67366,#67367,#67368));
#14985=EDGE_LOOP('',(#67369,#67370,#67371,#67372));
#14986=EDGE_LOOP('',(#67373,#67374,#67375,#67376));
#14987=EDGE_LOOP('',(#67377,#67378,#67379,#67380,#67381));
#14988=EDGE_LOOP('',(#67382,#67383,#67384,#67385));
#14989=EDGE_LOOP('',(#67386,#67387,#67388,#67389));
#14990=EDGE_LOOP('',(#67390,#67391,#67392,#67393));
#14991=EDGE_LOOP('',(#67394,#67395,#67396,#67397));
#14992=EDGE_LOOP('',(#67398,#67399,#67400,#67401,#67402));
#14993=EDGE_LOOP('',(#67403,#67404,#67405,#67406));
#14994=EDGE_LOOP('',(#67407,#67408,#67409,#67410));
#14995=EDGE_LOOP('',(#67411,#67412,#67413,#67414));
#14996=EDGE_LOOP('',(#67415,#67416,#67417,#67418));
#14997=EDGE_LOOP('',(#67419,#67420,#67421,#67422));
#14998=EDGE_LOOP('',(#67423,#67424,#67425,#67426));
#14999=EDGE_LOOP('',(#67427,#67428,#67429,#67430));
#15000=EDGE_LOOP('',(#67431,#67432,#67433,#67434));
#15001=EDGE_LOOP('',(#67435,#67436,#67437,#67438));
#15002=EDGE_LOOP('',(#67439,#67440,#67441,#67442));
#15003=EDGE_LOOP('',(#67443,#67444,#67445,#67446,#67447));
#15004=EDGE_LOOP('',(#67448,#67449,#67450,#67451));
#15005=EDGE_LOOP('',(#67452,#67453,#67454,#67455));
#15006=EDGE_LOOP('',(#67456,#67457,#67458,#67459));
#15007=EDGE_LOOP('',(#67460,#67461,#67462,#67463));
#15008=EDGE_LOOP('',(#67464,#67465,#67466,#67467));
#15009=EDGE_LOOP('',(#67468,#67469,#67470,#67471));
#15010=EDGE_LOOP('',(#67472,#67473,#67474,#67475));
#15011=EDGE_LOOP('',(#67476,#67477,#67478,#67479));
#15012=EDGE_LOOP('',(#67480,#67481,#67482,#67483,#67484));
#15013=EDGE_LOOP('',(#67485,#67486,#67487,#67488));
#15014=EDGE_LOOP('',(#67489,#67490,#67491,#67492));
#15015=EDGE_LOOP('',(#67493,#67494,#67495,#67496,#67497));
#15016=EDGE_LOOP('',(#67498,#67499,#67500,#67501));
#15017=EDGE_LOOP('',(#67502,#67503,#67504,#67505));
#15018=EDGE_LOOP('',(#67506,#67507,#67508,#67509));
#15019=EDGE_LOOP('',(#67510,#67511,#67512,#67513));
#15020=EDGE_LOOP('',(#67514,#67515,#67516,#67517,#67518));
#15021=EDGE_LOOP('',(#67519,#67520,#67521,#67522));
#15022=EDGE_LOOP('',(#67523,#67524,#67525,#67526));
#15023=EDGE_LOOP('',(#67527,#67528,#67529,#67530));
#15024=EDGE_LOOP('',(#67531,#67532,#67533,#67534));
#15025=EDGE_LOOP('',(#67535,#67536,#67537,#67538));
#15026=EDGE_LOOP('',(#67539,#67540,#67541,#67542));
#15027=EDGE_LOOP('',(#67543,#67544,#67545,#67546));
#15028=EDGE_LOOP('',(#67547,#67548,#67549,#67550));
#15029=EDGE_LOOP('',(#67551,#67552,#67553,#67554));
#15030=EDGE_LOOP('',(#67555,#67556,#67557,#67558));
#15031=EDGE_LOOP('',(#67559,#67560,#67561,#67562,#67563));
#15032=EDGE_LOOP('',(#67564,#67565,#67566,#67567));
#15033=EDGE_LOOP('',(#67568,#67569,#67570,#67571));
#15034=EDGE_LOOP('',(#67572,#67573,#67574,#67575));
#15035=EDGE_LOOP('',(#67576,#67577,#67578,#67579));
#15036=EDGE_LOOP('',(#67580,#67581,#67582,#67583));
#15037=EDGE_LOOP('',(#67584,#67585,#67586,#67587));
#15038=EDGE_LOOP('',(#67588,#67589,#67590,#67591));
#15039=EDGE_LOOP('',(#67592,#67593,#67594,#67595));
#15040=EDGE_LOOP('',(#67596,#67597,#67598,#67599,#67600));
#15041=EDGE_LOOP('',(#67601,#67602,#67603,#67604));
#15042=EDGE_LOOP('',(#67605,#67606,#67607,#67608));
#15043=EDGE_LOOP('',(#67609,#67610,#67611,#67612,#67613));
#15044=EDGE_LOOP('',(#67614,#67615,#67616,#67617));
#15045=EDGE_LOOP('',(#67618,#67619,#67620,#67621));
#15046=EDGE_LOOP('',(#67622,#67623,#67624,#67625));
#15047=EDGE_LOOP('',(#67626,#67627,#67628,#67629));
#15048=EDGE_LOOP('',(#67630,#67631,#67632,#67633,#67634));
#15049=EDGE_LOOP('',(#67635,#67636,#67637,#67638));
#15050=EDGE_LOOP('',(#67639,#67640,#67641,#67642));
#15051=EDGE_LOOP('',(#67643,#67644,#67645,#67646));
#15052=EDGE_LOOP('',(#67647,#67648,#67649,#67650));
#15053=EDGE_LOOP('',(#67651,#67652,#67653,#67654));
#15054=EDGE_LOOP('',(#67655,#67656,#67657,#67658));
#15055=EDGE_LOOP('',(#67659,#67660,#67661,#67662));
#15056=EDGE_LOOP('',(#67663,#67664,#67665,#67666));
#15057=EDGE_LOOP('',(#67667,#67668,#67669,#67670));
#15058=EDGE_LOOP('',(#67671,#67672,#67673,#67674));
#15059=EDGE_LOOP('',(#67675,#67676,#67677,#67678,#67679));
#15060=EDGE_LOOP('',(#67680,#67681,#67682,#67683));
#15061=EDGE_LOOP('',(#67684,#67685,#67686,#67687));
#15062=EDGE_LOOP('',(#67688,#67689,#67690,#67691));
#15063=EDGE_LOOP('',(#67692,#67693,#67694,#67695));
#15064=EDGE_LOOP('',(#67696,#67697,#67698,#67699));
#15065=EDGE_LOOP('',(#67700,#67701,#67702,#67703));
#15066=EDGE_LOOP('',(#67704,#67705,#67706,#67707));
#15067=EDGE_LOOP('',(#67708,#67709,#67710,#67711));
#15068=EDGE_LOOP('',(#67712,#67713,#67714,#67715,#67716));
#15069=EDGE_LOOP('',(#67717,#67718,#67719,#67720));
#15070=EDGE_LOOP('',(#67721,#67722,#67723,#67724));
#15071=EDGE_LOOP('',(#67725,#67726,#67727,#67728,#67729));
#15072=EDGE_LOOP('',(#67730,#67731,#67732,#67733));
#15073=EDGE_LOOP('',(#67734,#67735,#67736,#67737));
#15074=EDGE_LOOP('',(#67738,#67739,#67740,#67741));
#15075=EDGE_LOOP('',(#67742,#67743,#67744,#67745));
#15076=EDGE_LOOP('',(#67746,#67747,#67748,#67749,#67750));
#15077=EDGE_LOOP('',(#67751,#67752,#67753,#67754));
#15078=EDGE_LOOP('',(#67755,#67756,#67757,#67758));
#15079=EDGE_LOOP('',(#67759,#67760,#67761,#67762));
#15080=EDGE_LOOP('',(#67763,#67764,#67765,#67766));
#15081=EDGE_LOOP('',(#67767,#67768,#67769,#67770));
#15082=EDGE_LOOP('',(#67771,#67772,#67773,#67774));
#15083=EDGE_LOOP('',(#67775,#67776,#67777,#67778));
#15084=EDGE_LOOP('',(#67779,#67780,#67781,#67782));
#15085=EDGE_LOOP('',(#67783,#67784,#67785,#67786));
#15086=EDGE_LOOP('',(#67787,#67788,#67789,#67790));
#15087=EDGE_LOOP('',(#67791,#67792,#67793,#67794,#67795));
#15088=EDGE_LOOP('',(#67796,#67797,#67798,#67799));
#15089=EDGE_LOOP('',(#67800,#67801,#67802,#67803));
#15090=EDGE_LOOP('',(#67804,#67805,#67806,#67807));
#15091=EDGE_LOOP('',(#67808,#67809,#67810,#67811));
#15092=EDGE_LOOP('',(#67812,#67813,#67814,#67815));
#15093=EDGE_LOOP('',(#67816,#67817,#67818,#67819));
#15094=EDGE_LOOP('',(#67820,#67821,#67822,#67823));
#15095=EDGE_LOOP('',(#67824,#67825,#67826,#67827));
#15096=EDGE_LOOP('',(#67828,#67829,#67830,#67831,#67832));
#15097=EDGE_LOOP('',(#67833,#67834,#67835,#67836));
#15098=EDGE_LOOP('',(#67837,#67838,#67839,#67840));
#15099=EDGE_LOOP('',(#67841,#67842,#67843,#67844,#67845));
#15100=EDGE_LOOP('',(#67846,#67847,#67848,#67849));
#15101=EDGE_LOOP('',(#67850,#67851,#67852,#67853));
#15102=EDGE_LOOP('',(#67854,#67855,#67856,#67857));
#15103=EDGE_LOOP('',(#67858,#67859,#67860,#67861));
#15104=EDGE_LOOP('',(#67862,#67863,#67864,#67865,#67866));
#15105=EDGE_LOOP('',(#67867,#67868,#67869,#67870));
#15106=EDGE_LOOP('',(#67871,#67872,#67873,#67874));
#15107=EDGE_LOOP('',(#67875,#67876,#67877,#67878));
#15108=EDGE_LOOP('',(#67879,#67880,#67881,#67882));
#15109=EDGE_LOOP('',(#67883,#67884,#67885,#67886));
#15110=EDGE_LOOP('',(#67887,#67888,#67889,#67890));
#15111=EDGE_LOOP('',(#67891,#67892,#67893,#67894));
#15112=EDGE_LOOP('',(#67895,#67896,#67897,#67898));
#15113=EDGE_LOOP('',(#67899,#67900,#67901,#67902));
#15114=EDGE_LOOP('',(#67903,#67904,#67905,#67906));
#15115=EDGE_LOOP('',(#67907,#67908,#67909,#67910,#67911));
#15116=EDGE_LOOP('',(#67912,#67913,#67914,#67915));
#15117=EDGE_LOOP('',(#67916,#67917,#67918,#67919));
#15118=EDGE_LOOP('',(#67920,#67921,#67922,#67923));
#15119=EDGE_LOOP('',(#67924,#67925,#67926,#67927));
#15120=EDGE_LOOP('',(#67928,#67929,#67930,#67931));
#15121=EDGE_LOOP('',(#67932,#67933,#67934,#67935));
#15122=EDGE_LOOP('',(#67936,#67937,#67938,#67939));
#15123=EDGE_LOOP('',(#67940,#67941,#67942,#67943));
#15124=EDGE_LOOP('',(#67944,#67945,#67946,#67947,#67948));
#15125=EDGE_LOOP('',(#67949,#67950,#67951,#67952));
#15126=EDGE_LOOP('',(#67953,#67954,#67955,#67956));
#15127=EDGE_LOOP('',(#67957,#67958,#67959,#67960,#67961));
#15128=EDGE_LOOP('',(#67962,#67963,#67964,#67965));
#15129=EDGE_LOOP('',(#67966,#67967,#67968,#67969));
#15130=EDGE_LOOP('',(#67970,#67971,#67972,#67973));
#15131=EDGE_LOOP('',(#67974,#67975,#67976,#67977));
#15132=EDGE_LOOP('',(#67978,#67979,#67980,#67981,#67982));
#15133=EDGE_LOOP('',(#67983,#67984,#67985,#67986));
#15134=EDGE_LOOP('',(#67987,#67988,#67989,#67990));
#15135=EDGE_LOOP('',(#67991,#67992,#67993,#67994));
#15136=EDGE_LOOP('',(#67995,#67996,#67997,#67998));
#15137=EDGE_LOOP('',(#67999,#68000,#68001,#68002));
#15138=EDGE_LOOP('',(#68003,#68004,#68005,#68006));
#15139=EDGE_LOOP('',(#68007,#68008,#68009,#68010));
#15140=EDGE_LOOP('',(#68011,#68012,#68013,#68014));
#15141=EDGE_LOOP('',(#68015,#68016,#68017,#68018));
#15142=EDGE_LOOP('',(#68019,#68020,#68021,#68022));
#15143=EDGE_LOOP('',(#68023,#68024,#68025,#68026,#68027));
#15144=EDGE_LOOP('',(#68028,#68029,#68030,#68031));
#15145=EDGE_LOOP('',(#68032,#68033,#68034,#68035));
#15146=EDGE_LOOP('',(#68036,#68037,#68038,#68039));
#15147=EDGE_LOOP('',(#68040,#68041,#68042,#68043));
#15148=EDGE_LOOP('',(#68044,#68045,#68046,#68047));
#15149=EDGE_LOOP('',(#68048,#68049,#68050,#68051));
#15150=EDGE_LOOP('',(#68052,#68053,#68054,#68055));
#15151=EDGE_LOOP('',(#68056,#68057,#68058,#68059));
#15152=EDGE_LOOP('',(#68060,#68061,#68062,#68063,#68064));
#15153=EDGE_LOOP('',(#68065,#68066,#68067,#68068));
#15154=EDGE_LOOP('',(#68069,#68070,#68071,#68072));
#15155=EDGE_LOOP('',(#68073,#68074,#68075,#68076,#68077));
#15156=EDGE_LOOP('',(#68078,#68079,#68080,#68081));
#15157=EDGE_LOOP('',(#68082,#68083,#68084,#68085));
#15158=EDGE_LOOP('',(#68086,#68087,#68088,#68089));
#15159=EDGE_LOOP('',(#68090,#68091,#68092,#68093));
#15160=EDGE_LOOP('',(#68094,#68095,#68096,#68097,#68098));
#15161=EDGE_LOOP('',(#68099,#68100,#68101,#68102));
#15162=EDGE_LOOP('',(#68103,#68104,#68105,#68106));
#15163=EDGE_LOOP('',(#68107,#68108,#68109,#68110));
#15164=EDGE_LOOP('',(#68111,#68112,#68113,#68114));
#15165=EDGE_LOOP('',(#68115,#68116,#68117,#68118));
#15166=EDGE_LOOP('',(#68119,#68120,#68121,#68122));
#15167=EDGE_LOOP('',(#68123,#68124,#68125,#68126));
#15168=EDGE_LOOP('',(#68127,#68128,#68129,#68130));
#15169=EDGE_LOOP('',(#68131,#68132,#68133,#68134));
#15170=EDGE_LOOP('',(#68135,#68136,#68137,#68138));
#15171=EDGE_LOOP('',(#68139,#68140,#68141,#68142,#68143));
#15172=EDGE_LOOP('',(#68144,#68145,#68146,#68147));
#15173=EDGE_LOOP('',(#68148,#68149,#68150,#68151));
#15174=EDGE_LOOP('',(#68152,#68153,#68154,#68155));
#15175=EDGE_LOOP('',(#68156,#68157,#68158,#68159));
#15176=EDGE_LOOP('',(#68160,#68161,#68162,#68163));
#15177=EDGE_LOOP('',(#68164,#68165,#68166,#68167));
#15178=EDGE_LOOP('',(#68168,#68169,#68170,#68171));
#15179=EDGE_LOOP('',(#68172,#68173,#68174,#68175));
#15180=EDGE_LOOP('',(#68176,#68177,#68178,#68179,#68180));
#15181=EDGE_LOOP('',(#68181,#68182,#68183,#68184));
#15182=EDGE_LOOP('',(#68185,#68186,#68187,#68188));
#15183=EDGE_LOOP('',(#68189,#68190,#68191,#68192,#68193));
#15184=EDGE_LOOP('',(#68194,#68195,#68196,#68197));
#15185=EDGE_LOOP('',(#68198,#68199,#68200,#68201));
#15186=EDGE_LOOP('',(#68202,#68203,#68204,#68205));
#15187=EDGE_LOOP('',(#68206,#68207,#68208,#68209));
#15188=EDGE_LOOP('',(#68210,#68211,#68212,#68213,#68214));
#15189=EDGE_LOOP('',(#68215,#68216,#68217,#68218));
#15190=EDGE_LOOP('',(#68219,#68220,#68221,#68222));
#15191=EDGE_LOOP('',(#68223,#68224,#68225,#68226));
#15192=EDGE_LOOP('',(#68227,#68228,#68229,#68230));
#15193=EDGE_LOOP('',(#68231,#68232,#68233,#68234));
#15194=EDGE_LOOP('',(#68235,#68236,#68237,#68238));
#15195=EDGE_LOOP('',(#68239,#68240,#68241,#68242));
#15196=EDGE_LOOP('',(#68243,#68244,#68245,#68246));
#15197=EDGE_LOOP('',(#68247,#68248,#68249,#68250));
#15198=EDGE_LOOP('',(#68251,#68252,#68253,#68254));
#15199=EDGE_LOOP('',(#68255,#68256,#68257,#68258,#68259));
#15200=EDGE_LOOP('',(#68260,#68261,#68262,#68263));
#15201=EDGE_LOOP('',(#68264,#68265,#68266,#68267));
#15202=EDGE_LOOP('',(#68268,#68269,#68270,#68271));
#15203=EDGE_LOOP('',(#68272,#68273,#68274,#68275));
#15204=EDGE_LOOP('',(#68276,#68277,#68278,#68279));
#15205=EDGE_LOOP('',(#68280,#68281,#68282,#68283));
#15206=EDGE_LOOP('',(#68284,#68285,#68286,#68287));
#15207=EDGE_LOOP('',(#68288,#68289,#68290,#68291));
#15208=EDGE_LOOP('',(#68292,#68293,#68294,#68295,#68296));
#15209=EDGE_LOOP('',(#68297,#68298,#68299,#68300));
#15210=EDGE_LOOP('',(#68301,#68302,#68303,#68304));
#15211=EDGE_LOOP('',(#68305,#68306,#68307,#68308,#68309));
#15212=EDGE_LOOP('',(#68310,#68311,#68312,#68313));
#15213=EDGE_LOOP('',(#68314,#68315,#68316,#68317));
#15214=EDGE_LOOP('',(#68318,#68319,#68320,#68321));
#15215=EDGE_LOOP('',(#68322,#68323,#68324,#68325));
#15216=EDGE_LOOP('',(#68326,#68327,#68328,#68329,#68330));
#15217=EDGE_LOOP('',(#68331,#68332,#68333,#68334));
#15218=EDGE_LOOP('',(#68335,#68336,#68337,#68338));
#15219=EDGE_LOOP('',(#68339,#68340,#68341,#68342));
#15220=EDGE_LOOP('',(#68343,#68344,#68345,#68346));
#15221=EDGE_LOOP('',(#68347,#68348,#68349,#68350));
#15222=EDGE_LOOP('',(#68351,#68352,#68353,#68354));
#15223=EDGE_LOOP('',(#68355,#68356,#68357,#68358));
#15224=EDGE_LOOP('',(#68359,#68360,#68361,#68362));
#15225=EDGE_LOOP('',(#68363,#68364,#68365,#68366));
#15226=EDGE_LOOP('',(#68367,#68368,#68369,#68370));
#15227=EDGE_LOOP('',(#68371,#68372,#68373,#68374,#68375));
#15228=EDGE_LOOP('',(#68376,#68377,#68378,#68379));
#15229=EDGE_LOOP('',(#68380,#68381,#68382,#68383));
#15230=EDGE_LOOP('',(#68384,#68385,#68386,#68387));
#15231=EDGE_LOOP('',(#68388,#68389,#68390,#68391));
#15232=EDGE_LOOP('',(#68392,#68393,#68394,#68395));
#15233=EDGE_LOOP('',(#68396,#68397,#68398,#68399));
#15234=EDGE_LOOP('',(#68400,#68401,#68402,#68403));
#15235=EDGE_LOOP('',(#68404,#68405,#68406,#68407));
#15236=EDGE_LOOP('',(#68408,#68409,#68410,#68411,#68412));
#15237=EDGE_LOOP('',(#68413,#68414,#68415,#68416));
#15238=EDGE_LOOP('',(#68417,#68418,#68419,#68420));
#15239=EDGE_LOOP('',(#68421,#68422,#68423,#68424,#68425));
#15240=EDGE_LOOP('',(#68426,#68427,#68428,#68429));
#15241=EDGE_LOOP('',(#68430,#68431,#68432,#68433));
#15242=EDGE_LOOP('',(#68434,#68435,#68436,#68437));
#15243=EDGE_LOOP('',(#68438,#68439,#68440,#68441));
#15244=EDGE_LOOP('',(#68442,#68443,#68444,#68445,#68446));
#15245=EDGE_LOOP('',(#68447,#68448,#68449,#68450));
#15246=EDGE_LOOP('',(#68451,#68452,#68453,#68454));
#15247=EDGE_LOOP('',(#68455,#68456,#68457,#68458));
#15248=EDGE_LOOP('',(#68459,#68460,#68461,#68462));
#15249=EDGE_LOOP('',(#68463,#68464,#68465,#68466));
#15250=EDGE_LOOP('',(#68467,#68468,#68469,#68470));
#15251=EDGE_LOOP('',(#68471,#68472,#68473,#68474));
#15252=EDGE_LOOP('',(#68475,#68476,#68477,#68478));
#15253=EDGE_LOOP('',(#68479,#68480,#68481,#68482));
#15254=EDGE_LOOP('',(#68483,#68484,#68485,#68486));
#15255=EDGE_LOOP('',(#68487,#68488,#68489,#68490,#68491));
#15256=EDGE_LOOP('',(#68492,#68493,#68494,#68495));
#15257=EDGE_LOOP('',(#68496,#68497,#68498,#68499));
#15258=EDGE_LOOP('',(#68500,#68501,#68502,#68503));
#15259=EDGE_LOOP('',(#68504,#68505,#68506,#68507));
#15260=EDGE_LOOP('',(#68508,#68509,#68510,#68511));
#15261=EDGE_LOOP('',(#68512,#68513,#68514,#68515));
#15262=EDGE_LOOP('',(#68516,#68517,#68518,#68519));
#15263=EDGE_LOOP('',(#68520,#68521,#68522,#68523));
#15264=EDGE_LOOP('',(#68524,#68525,#68526,#68527,#68528));
#15265=EDGE_LOOP('',(#68529,#68530,#68531,#68532));
#15266=EDGE_LOOP('',(#68533,#68534,#68535,#68536));
#15267=EDGE_LOOP('',(#68537,#68538,#68539,#68540,#68541));
#15268=EDGE_LOOP('',(#68542,#68543,#68544,#68545));
#15269=EDGE_LOOP('',(#68546,#68547,#68548,#68549));
#15270=EDGE_LOOP('',(#68550,#68551,#68552,#68553));
#15271=EDGE_LOOP('',(#68554,#68555,#68556,#68557));
#15272=EDGE_LOOP('',(#68558,#68559,#68560,#68561,#68562));
#15273=EDGE_LOOP('',(#68563,#68564,#68565,#68566));
#15274=EDGE_LOOP('',(#68567,#68568,#68569,#68570));
#15275=EDGE_LOOP('',(#68571,#68572,#68573,#68574));
#15276=EDGE_LOOP('',(#68575,#68576,#68577,#68578));
#15277=EDGE_LOOP('',(#68579,#68580,#68581,#68582));
#15278=EDGE_LOOP('',(#68583,#68584,#68585,#68586));
#15279=EDGE_LOOP('',(#68587,#68588,#68589,#68590));
#15280=EDGE_LOOP('',(#68591,#68592,#68593,#68594));
#15281=EDGE_LOOP('',(#68595,#68596,#68597,#68598));
#15282=EDGE_LOOP('',(#68599,#68600,#68601,#68602));
#15283=EDGE_LOOP('',(#68603,#68604,#68605,#68606,#68607));
#15284=EDGE_LOOP('',(#68608,#68609,#68610,#68611));
#15285=EDGE_LOOP('',(#68612,#68613,#68614,#68615));
#15286=EDGE_LOOP('',(#68616,#68617,#68618,#68619));
#15287=EDGE_LOOP('',(#68620,#68621,#68622,#68623));
#15288=EDGE_LOOP('',(#68624,#68625,#68626,#68627));
#15289=EDGE_LOOP('',(#68628,#68629,#68630,#68631));
#15290=EDGE_LOOP('',(#68632,#68633,#68634,#68635));
#15291=EDGE_LOOP('',(#68636,#68637,#68638,#68639));
#15292=EDGE_LOOP('',(#68640,#68641,#68642,#68643,#68644));
#15293=EDGE_LOOP('',(#68645,#68646,#68647,#68648));
#15294=EDGE_LOOP('',(#68649,#68650,#68651,#68652));
#15295=EDGE_LOOP('',(#68653,#68654,#68655,#68656,#68657));
#15296=EDGE_LOOP('',(#68658,#68659,#68660,#68661));
#15297=EDGE_LOOP('',(#68662,#68663,#68664,#68665));
#15298=EDGE_LOOP('',(#68666,#68667,#68668,#68669));
#15299=EDGE_LOOP('',(#68670,#68671,#68672,#68673));
#15300=EDGE_LOOP('',(#68674,#68675,#68676,#68677,#68678));
#15301=EDGE_LOOP('',(#68679,#68680,#68681,#68682));
#15302=EDGE_LOOP('',(#68683,#68684,#68685,#68686));
#15303=EDGE_LOOP('',(#68687,#68688,#68689,#68690));
#15304=EDGE_LOOP('',(#68691,#68692,#68693,#68694));
#15305=EDGE_LOOP('',(#68695,#68696,#68697,#68698));
#15306=EDGE_LOOP('',(#68699,#68700,#68701,#68702));
#15307=EDGE_LOOP('',(#68703,#68704,#68705,#68706));
#15308=EDGE_LOOP('',(#68707,#68708,#68709,#68710));
#15309=EDGE_LOOP('',(#68711,#68712,#68713,#68714));
#15310=EDGE_LOOP('',(#68715,#68716,#68717,#68718));
#15311=EDGE_LOOP('',(#68719,#68720,#68721,#68722,#68723));
#15312=EDGE_LOOP('',(#68724,#68725,#68726,#68727));
#15313=EDGE_LOOP('',(#68728,#68729,#68730,#68731));
#15314=EDGE_LOOP('',(#68732,#68733,#68734,#68735));
#15315=EDGE_LOOP('',(#68736,#68737,#68738,#68739));
#15316=EDGE_LOOP('',(#68740,#68741,#68742,#68743));
#15317=EDGE_LOOP('',(#68744,#68745,#68746,#68747));
#15318=EDGE_LOOP('',(#68748,#68749,#68750,#68751));
#15319=EDGE_LOOP('',(#68752,#68753,#68754,#68755));
#15320=EDGE_LOOP('',(#68756,#68757,#68758,#68759,#68760));
#15321=EDGE_LOOP('',(#68761,#68762,#68763,#68764));
#15322=EDGE_LOOP('',(#68765,#68766,#68767,#68768));
#15323=EDGE_LOOP('',(#68769,#68770,#68771,#68772,#68773));
#15324=EDGE_LOOP('',(#68774,#68775,#68776,#68777));
#15325=EDGE_LOOP('',(#68778,#68779,#68780,#68781));
#15326=EDGE_LOOP('',(#68782,#68783,#68784,#68785));
#15327=EDGE_LOOP('',(#68786,#68787,#68788,#68789));
#15328=EDGE_LOOP('',(#68790,#68791,#68792,#68793,#68794));
#15329=EDGE_LOOP('',(#68795,#68796,#68797,#68798));
#15330=EDGE_LOOP('',(#68799,#68800,#68801,#68802));
#15331=EDGE_LOOP('',(#68803,#68804,#68805,#68806));
#15332=EDGE_LOOP('',(#68807,#68808,#68809,#68810));
#15333=EDGE_LOOP('',(#68811,#68812,#68813,#68814));
#15334=EDGE_LOOP('',(#68815,#68816,#68817,#68818));
#15335=EDGE_LOOP('',(#68819,#68820,#68821,#68822));
#15336=EDGE_LOOP('',(#68823,#68824,#68825,#68826));
#15337=EDGE_LOOP('',(#68827,#68828,#68829,#68830));
#15338=EDGE_LOOP('',(#68831,#68832,#68833,#68834));
#15339=EDGE_LOOP('',(#68835,#68836,#68837,#68838,#68839));
#15340=EDGE_LOOP('',(#68840,#68841,#68842,#68843));
#15341=EDGE_LOOP('',(#68844,#68845,#68846,#68847));
#15342=EDGE_LOOP('',(#68848,#68849,#68850,#68851));
#15343=EDGE_LOOP('',(#68852,#68853,#68854,#68855));
#15344=EDGE_LOOP('',(#68856,#68857,#68858,#68859));
#15345=EDGE_LOOP('',(#68860,#68861,#68862,#68863));
#15346=EDGE_LOOP('',(#68864,#68865,#68866,#68867));
#15347=EDGE_LOOP('',(#68868,#68869,#68870,#68871));
#15348=EDGE_LOOP('',(#68872,#68873,#68874,#68875,#68876));
#15349=EDGE_LOOP('',(#68877,#68878,#68879,#68880));
#15350=EDGE_LOOP('',(#68881,#68882,#68883,#68884));
#15351=EDGE_LOOP('',(#68885,#68886,#68887,#68888,#68889));
#15352=EDGE_LOOP('',(#68890,#68891,#68892,#68893));
#15353=EDGE_LOOP('',(#68894,#68895,#68896,#68897));
#15354=EDGE_LOOP('',(#68898,#68899,#68900,#68901));
#15355=EDGE_LOOP('',(#68902,#68903,#68904,#68905));
#15356=EDGE_LOOP('',(#68906,#68907,#68908,#68909,#68910));
#15357=EDGE_LOOP('',(#68911,#68912,#68913,#68914));
#15358=EDGE_LOOP('',(#68915,#68916,#68917,#68918));
#15359=EDGE_LOOP('',(#68919,#68920,#68921,#68922));
#15360=EDGE_LOOP('',(#68923,#68924,#68925,#68926));
#15361=EDGE_LOOP('',(#68927,#68928,#68929,#68930));
#15362=EDGE_LOOP('',(#68931,#68932,#68933,#68934));
#15363=EDGE_LOOP('',(#68935,#68936,#68937,#68938));
#15364=EDGE_LOOP('',(#68939,#68940,#68941,#68942));
#15365=EDGE_LOOP('',(#68943,#68944,#68945,#68946));
#15366=EDGE_LOOP('',(#68947,#68948,#68949,#68950));
#15367=EDGE_LOOP('',(#68951,#68952,#68953,#68954,#68955));
#15368=EDGE_LOOP('',(#68956,#68957,#68958,#68959));
#15369=EDGE_LOOP('',(#68960,#68961,#68962,#68963));
#15370=EDGE_LOOP('',(#68964,#68965,#68966,#68967));
#15371=EDGE_LOOP('',(#68968,#68969,#68970,#68971));
#15372=EDGE_LOOP('',(#68972,#68973,#68974,#68975));
#15373=EDGE_LOOP('',(#68976,#68977,#68978,#68979));
#15374=EDGE_LOOP('',(#68980,#68981,#68982,#68983));
#15375=EDGE_LOOP('',(#68984,#68985,#68986,#68987));
#15376=EDGE_LOOP('',(#68988,#68989,#68990,#68991,#68992));
#15377=EDGE_LOOP('',(#68993,#68994,#68995,#68996));
#15378=EDGE_LOOP('',(#68997,#68998,#68999,#69000));
#15379=EDGE_LOOP('',(#69001,#69002,#69003,#69004,#69005));
#15380=EDGE_LOOP('',(#69006,#69007,#69008,#69009));
#15381=EDGE_LOOP('',(#69010,#69011,#69012,#69013));
#15382=EDGE_LOOP('',(#69014,#69015,#69016,#69017));
#15383=EDGE_LOOP('',(#69018,#69019,#69020,#69021));
#15384=EDGE_LOOP('',(#69022,#69023,#69024,#69025,#69026));
#15385=EDGE_LOOP('',(#69027,#69028,#69029,#69030));
#15386=EDGE_LOOP('',(#69031,#69032,#69033,#69034));
#15387=EDGE_LOOP('',(#69035,#69036,#69037,#69038));
#15388=EDGE_LOOP('',(#69039,#69040,#69041,#69042));
#15389=EDGE_LOOP('',(#69043,#69044,#69045,#69046));
#15390=EDGE_LOOP('',(#69047,#69048,#69049,#69050));
#15391=EDGE_LOOP('',(#69051,#69052,#69053,#69054));
#15392=EDGE_LOOP('',(#69055,#69056,#69057,#69058));
#15393=EDGE_LOOP('',(#69059,#69060,#69061,#69062));
#15394=EDGE_LOOP('',(#69063,#69064,#69065,#69066));
#15395=EDGE_LOOP('',(#69067,#69068,#69069,#69070,#69071));
#15396=EDGE_LOOP('',(#69072,#69073,#69074,#69075));
#15397=EDGE_LOOP('',(#69076,#69077,#69078,#69079));
#15398=EDGE_LOOP('',(#69080,#69081,#69082,#69083));
#15399=EDGE_LOOP('',(#69084,#69085,#69086,#69087));
#15400=EDGE_LOOP('',(#69088,#69089,#69090,#69091));
#15401=EDGE_LOOP('',(#69092,#69093,#69094,#69095));
#15402=EDGE_LOOP('',(#69096,#69097,#69098,#69099));
#15403=EDGE_LOOP('',(#69100,#69101,#69102,#69103));
#15404=EDGE_LOOP('',(#69104,#69105,#69106,#69107,#69108));
#15405=EDGE_LOOP('',(#69109,#69110,#69111,#69112));
#15406=EDGE_LOOP('',(#69113,#69114,#69115,#69116));
#15407=EDGE_LOOP('',(#69117,#69118,#69119,#69120,#69121));
#15408=EDGE_LOOP('',(#69122,#69123,#69124,#69125));
#15409=EDGE_LOOP('',(#69126,#69127,#69128,#69129));
#15410=EDGE_LOOP('',(#69130,#69131,#69132,#69133));
#15411=EDGE_LOOP('',(#69134,#69135,#69136,#69137));
#15412=EDGE_LOOP('',(#69138,#69139,#69140,#69141,#69142));
#15413=EDGE_LOOP('',(#69143,#69144,#69145,#69146));
#15414=EDGE_LOOP('',(#69147,#69148,#69149,#69150));
#15415=EDGE_LOOP('',(#69151,#69152,#69153,#69154));
#15416=EDGE_LOOP('',(#69155,#69156,#69157,#69158));
#15417=EDGE_LOOP('',(#69159,#69160,#69161,#69162));
#15418=EDGE_LOOP('',(#69163,#69164,#69165,#69166));
#15419=EDGE_LOOP('',(#69167,#69168,#69169,#69170));
#15420=EDGE_LOOP('',(#69171,#69172,#69173,#69174));
#15421=EDGE_LOOP('',(#69175,#69176,#69177,#69178));
#15422=EDGE_LOOP('',(#69179,#69180,#69181,#69182));
#15423=EDGE_LOOP('',(#69183,#69184,#69185,#69186,#69187));
#15424=EDGE_LOOP('',(#69188,#69189,#69190,#69191));
#15425=EDGE_LOOP('',(#69192,#69193,#69194,#69195));
#15426=EDGE_LOOP('',(#69196,#69197,#69198,#69199));
#15427=EDGE_LOOP('',(#69200,#69201,#69202,#69203));
#15428=EDGE_LOOP('',(#69204,#69205,#69206,#69207));
#15429=EDGE_LOOP('',(#69208,#69209,#69210,#69211));
#15430=EDGE_LOOP('',(#69212,#69213,#69214,#69215));
#15431=EDGE_LOOP('',(#69216,#69217,#69218,#69219));
#15432=EDGE_LOOP('',(#69220,#69221,#69222,#69223,#69224));
#15433=EDGE_LOOP('',(#69225,#69226,#69227,#69228));
#15434=EDGE_LOOP('',(#69229,#69230,#69231,#69232));
#15435=EDGE_LOOP('',(#69233,#69234,#69235,#69236,#69237));
#15436=EDGE_LOOP('',(#69238,#69239,#69240,#69241));
#15437=EDGE_LOOP('',(#69242,#69243,#69244,#69245));
#15438=EDGE_LOOP('',(#69246,#69247,#69248,#69249));
#15439=EDGE_LOOP('',(#69250,#69251,#69252,#69253));
#15440=EDGE_LOOP('',(#69254,#69255,#69256,#69257,#69258));
#15441=EDGE_LOOP('',(#69259,#69260,#69261,#69262));
#15442=EDGE_LOOP('',(#69263,#69264,#69265,#69266));
#15443=EDGE_LOOP('',(#69267,#69268,#69269,#69270));
#15444=EDGE_LOOP('',(#69271,#69272,#69273,#69274));
#15445=EDGE_LOOP('',(#69275,#69276,#69277,#69278));
#15446=EDGE_LOOP('',(#69279,#69280,#69281,#69282));
#15447=EDGE_LOOP('',(#69283,#69284,#69285,#69286));
#15448=EDGE_LOOP('',(#69287,#69288,#69289,#69290));
#15449=EDGE_LOOP('',(#69291,#69292,#69293,#69294));
#15450=EDGE_LOOP('',(#69295,#69296,#69297,#69298));
#15451=EDGE_LOOP('',(#69299,#69300,#69301,#69302,#69303));
#15452=EDGE_LOOP('',(#69304,#69305,#69306,#69307));
#15453=EDGE_LOOP('',(#69308,#69309,#69310,#69311));
#15454=EDGE_LOOP('',(#69312,#69313,#69314,#69315));
#15455=EDGE_LOOP('',(#69316,#69317,#69318,#69319));
#15456=EDGE_LOOP('',(#69320,#69321,#69322,#69323));
#15457=EDGE_LOOP('',(#69324,#69325,#69326,#69327));
#15458=EDGE_LOOP('',(#69328,#69329,#69330,#69331));
#15459=EDGE_LOOP('',(#69332,#69333,#69334,#69335));
#15460=EDGE_LOOP('',(#69336,#69337,#69338,#69339,#69340));
#15461=EDGE_LOOP('',(#69341,#69342,#69343,#69344));
#15462=EDGE_LOOP('',(#69345,#69346,#69347,#69348));
#15463=EDGE_LOOP('',(#69349,#69350,#69351,#69352,#69353));
#15464=EDGE_LOOP('',(#69354,#69355,#69356,#69357));
#15465=EDGE_LOOP('',(#69358,#69359,#69360,#69361));
#15466=EDGE_LOOP('',(#69362,#69363,#69364,#69365));
#15467=EDGE_LOOP('',(#69366,#69367,#69368,#69369));
#15468=EDGE_LOOP('',(#69370,#69371,#69372,#69373,#69374));
#15469=EDGE_LOOP('',(#69375,#69376,#69377,#69378));
#15470=EDGE_LOOP('',(#69379,#69380,#69381,#69382));
#15471=EDGE_LOOP('',(#69383,#69384,#69385,#69386));
#15472=EDGE_LOOP('',(#69387,#69388,#69389,#69390));
#15473=EDGE_LOOP('',(#69391,#69392,#69393,#69394));
#15474=EDGE_LOOP('',(#69395,#69396,#69397,#69398));
#15475=EDGE_LOOP('',(#69399,#69400,#69401,#69402));
#15476=EDGE_LOOP('',(#69403,#69404,#69405,#69406));
#15477=EDGE_LOOP('',(#69407,#69408,#69409,#69410));
#15478=EDGE_LOOP('',(#69411,#69412,#69413,#69414));
#15479=EDGE_LOOP('',(#69415,#69416,#69417,#69418,#69419));
#15480=EDGE_LOOP('',(#69420,#69421,#69422,#69423));
#15481=EDGE_LOOP('',(#69424,#69425,#69426,#69427));
#15482=EDGE_LOOP('',(#69428,#69429,#69430,#69431));
#15483=EDGE_LOOP('',(#69432,#69433,#69434,#69435));
#15484=EDGE_LOOP('',(#69436,#69437,#69438,#69439));
#15485=EDGE_LOOP('',(#69440,#69441,#69442,#69443));
#15486=EDGE_LOOP('',(#69444,#69445,#69446,#69447));
#15487=EDGE_LOOP('',(#69448,#69449,#69450,#69451));
#15488=EDGE_LOOP('',(#69452,#69453,#69454,#69455,#69456));
#15489=EDGE_LOOP('',(#69457,#69458,#69459,#69460));
#15490=EDGE_LOOP('',(#69461,#69462,#69463,#69464));
#15491=EDGE_LOOP('',(#69465,#69466,#69467,#69468,#69469));
#15492=EDGE_LOOP('',(#69470,#69471,#69472,#69473));
#15493=EDGE_LOOP('',(#69474,#69475,#69476,#69477));
#15494=EDGE_LOOP('',(#69478,#69479,#69480,#69481));
#15495=EDGE_LOOP('',(#69482,#69483,#69484,#69485));
#15496=EDGE_LOOP('',(#69486,#69487,#69488,#69489,#69490));
#15497=EDGE_LOOP('',(#69491,#69492,#69493,#69494));
#15498=EDGE_LOOP('',(#69495,#69496,#69497,#69498));
#15499=EDGE_LOOP('',(#69499,#69500,#69501,#69502));
#15500=EDGE_LOOP('',(#69503,#69504,#69505,#69506));
#15501=EDGE_LOOP('',(#69507,#69508,#69509,#69510));
#15502=EDGE_LOOP('',(#69511,#69512,#69513,#69514));
#15503=EDGE_LOOP('',(#69515,#69516,#69517,#69518));
#15504=EDGE_LOOP('',(#69519,#69520,#69521,#69522));
#15505=EDGE_LOOP('',(#69523,#69524,#69525,#69526));
#15506=EDGE_LOOP('',(#69527,#69528,#69529,#69530));
#15507=EDGE_LOOP('',(#69531,#69532,#69533,#69534,#69535));
#15508=EDGE_LOOP('',(#69536,#69537,#69538,#69539));
#15509=EDGE_LOOP('',(#69540,#69541,#69542,#69543));
#15510=EDGE_LOOP('',(#69544,#69545,#69546,#69547));
#15511=EDGE_LOOP('',(#69548,#69549,#69550,#69551));
#15512=EDGE_LOOP('',(#69552,#69553,#69554,#69555));
#15513=EDGE_LOOP('',(#69556,#69557,#69558,#69559));
#15514=EDGE_LOOP('',(#69560,#69561,#69562,#69563));
#15515=EDGE_LOOP('',(#69564,#69565,#69566,#69567));
#15516=EDGE_LOOP('',(#69568,#69569,#69570,#69571,#69572));
#15517=EDGE_LOOP('',(#69573,#69574,#69575,#69576));
#15518=EDGE_LOOP('',(#69577,#69578,#69579,#69580));
#15519=EDGE_LOOP('',(#69581,#69582,#69583,#69584,#69585));
#15520=EDGE_LOOP('',(#69586,#69587,#69588,#69589));
#15521=EDGE_LOOP('',(#69590,#69591,#69592,#69593));
#15522=EDGE_LOOP('',(#69594,#69595,#69596,#69597));
#15523=EDGE_LOOP('',(#69598,#69599,#69600,#69601));
#15524=EDGE_LOOP('',(#69602,#69603,#69604,#69605,#69606));
#15525=EDGE_LOOP('',(#69607,#69608,#69609,#69610));
#15526=EDGE_LOOP('',(#69611,#69612,#69613,#69614));
#15527=EDGE_LOOP('',(#69615,#69616,#69617,#69618));
#15528=EDGE_LOOP('',(#69619,#69620,#69621,#69622));
#15529=EDGE_LOOP('',(#69623,#69624,#69625,#69626));
#15530=EDGE_LOOP('',(#69627,#69628,#69629,#69630));
#15531=EDGE_LOOP('',(#69631,#69632,#69633,#69634));
#15532=EDGE_LOOP('',(#69635,#69636,#69637,#69638));
#15533=EDGE_LOOP('',(#69639,#69640,#69641,#69642));
#15534=EDGE_LOOP('',(#69643,#69644,#69645,#69646));
#15535=EDGE_LOOP('',(#69647,#69648,#69649,#69650,#69651));
#15536=EDGE_LOOP('',(#69652,#69653,#69654,#69655));
#15537=EDGE_LOOP('',(#69656,#69657,#69658,#69659));
#15538=EDGE_LOOP('',(#69660,#69661,#69662,#69663));
#15539=EDGE_LOOP('',(#69664,#69665,#69666,#69667));
#15540=EDGE_LOOP('',(#69668,#69669,#69670,#69671));
#15541=EDGE_LOOP('',(#69672,#69673,#69674,#69675));
#15542=EDGE_LOOP('',(#69676,#69677,#69678,#69679));
#15543=EDGE_LOOP('',(#69680,#69681,#69682,#69683));
#15544=EDGE_LOOP('',(#69684,#69685,#69686,#69687,#69688));
#15545=EDGE_LOOP('',(#69689,#69690,#69691,#69692));
#15546=EDGE_LOOP('',(#69693,#69694,#69695,#69696));
#15547=EDGE_LOOP('',(#69697,#69698,#69699,#69700,#69701));
#15548=EDGE_LOOP('',(#69702,#69703,#69704,#69705));
#15549=EDGE_LOOP('',(#69706,#69707,#69708,#69709));
#15550=EDGE_LOOP('',(#69710,#69711,#69712,#69713));
#15551=EDGE_LOOP('',(#69714,#69715,#69716,#69717));
#15552=EDGE_LOOP('',(#69718,#69719,#69720,#69721,#69722));
#15553=EDGE_LOOP('',(#69723,#69724,#69725,#69726));
#15554=EDGE_LOOP('',(#69727,#69728,#69729,#69730));
#15555=EDGE_LOOP('',(#69731,#69732,#69733,#69734));
#15556=EDGE_LOOP('',(#69735,#69736,#69737,#69738));
#15557=EDGE_LOOP('',(#69739,#69740,#69741,#69742));
#15558=EDGE_LOOP('',(#69743,#69744,#69745,#69746));
#15559=EDGE_LOOP('',(#69747,#69748,#69749,#69750));
#15560=EDGE_LOOP('',(#69751,#69752,#69753,#69754));
#15561=EDGE_LOOP('',(#69755,#69756,#69757,#69758));
#15562=EDGE_LOOP('',(#69759,#69760,#69761,#69762));
#15563=EDGE_LOOP('',(#69763,#69764,#69765,#69766,#69767));
#15564=EDGE_LOOP('',(#69768,#69769,#69770,#69771));
#15565=EDGE_LOOP('',(#69772,#69773,#69774,#69775));
#15566=EDGE_LOOP('',(#69776,#69777,#69778,#69779));
#15567=EDGE_LOOP('',(#69780,#69781,#69782,#69783));
#15568=EDGE_LOOP('',(#69784,#69785,#69786,#69787));
#15569=EDGE_LOOP('',(#69788,#69789,#69790,#69791));
#15570=EDGE_LOOP('',(#69792,#69793,#69794,#69795));
#15571=EDGE_LOOP('',(#69796,#69797,#69798,#69799));
#15572=EDGE_LOOP('',(#69800,#69801,#69802,#69803,#69804));
#15573=EDGE_LOOP('',(#69805,#69806,#69807,#69808));
#15574=EDGE_LOOP('',(#69809,#69810,#69811,#69812));
#15575=EDGE_LOOP('',(#69813,#69814,#69815,#69816,#69817));
#15576=EDGE_LOOP('',(#69818,#69819,#69820,#69821));
#15577=EDGE_LOOP('',(#69822,#69823,#69824,#69825));
#15578=EDGE_LOOP('',(#69826,#69827,#69828,#69829));
#15579=EDGE_LOOP('',(#69830,#69831,#69832,#69833));
#15580=EDGE_LOOP('',(#69834,#69835,#69836,#69837,#69838));
#15581=EDGE_LOOP('',(#69839,#69840,#69841,#69842));
#15582=EDGE_LOOP('',(#69843,#69844,#69845,#69846));
#15583=EDGE_LOOP('',(#69847,#69848,#69849,#69850));
#15584=EDGE_LOOP('',(#69851,#69852,#69853,#69854));
#15585=EDGE_LOOP('',(#69855,#69856,#69857,#69858));
#15586=EDGE_LOOP('',(#69859,#69860,#69861,#69862));
#15587=EDGE_LOOP('',(#69863,#69864,#69865,#69866));
#15588=EDGE_LOOP('',(#69867,#69868,#69869,#69870));
#15589=EDGE_LOOP('',(#69871,#69872,#69873,#69874));
#15590=EDGE_LOOP('',(#69875,#69876,#69877,#69878));
#15591=EDGE_LOOP('',(#69879,#69880,#69881,#69882,#69883));
#15592=EDGE_LOOP('',(#69884,#69885,#69886,#69887));
#15593=EDGE_LOOP('',(#69888,#69889,#69890,#69891));
#15594=EDGE_LOOP('',(#69892,#69893,#69894,#69895));
#15595=EDGE_LOOP('',(#69896,#69897,#69898,#69899));
#15596=EDGE_LOOP('',(#69900,#69901,#69902,#69903));
#15597=EDGE_LOOP('',(#69904,#69905,#69906,#69907));
#15598=EDGE_LOOP('',(#69908,#69909,#69910,#69911));
#15599=EDGE_LOOP('',(#69912,#69913,#69914,#69915));
#15600=EDGE_LOOP('',(#69916,#69917,#69918,#69919,#69920));
#15601=EDGE_LOOP('',(#69921,#69922,#69923,#69924));
#15602=EDGE_LOOP('',(#69925,#69926,#69927,#69928));
#15603=EDGE_LOOP('',(#69929,#69930,#69931,#69932,#69933));
#15604=EDGE_LOOP('',(#69934,#69935,#69936,#69937));
#15605=EDGE_LOOP('',(#69938,#69939,#69940,#69941));
#15606=EDGE_LOOP('',(#69942,#69943,#69944,#69945));
#15607=EDGE_LOOP('',(#69946,#69947,#69948,#69949));
#15608=EDGE_LOOP('',(#69950,#69951,#69952,#69953,#69954));
#15609=EDGE_LOOP('',(#69955,#69956,#69957,#69958));
#15610=EDGE_LOOP('',(#69959,#69960,#69961,#69962));
#15611=EDGE_LOOP('',(#69963,#69964,#69965,#69966));
#15612=EDGE_LOOP('',(#69967,#69968,#69969,#69970));
#15613=EDGE_LOOP('',(#69971,#69972,#69973,#69974));
#15614=EDGE_LOOP('',(#69975,#69976,#69977,#69978));
#15615=EDGE_LOOP('',(#69979,#69980,#69981,#69982));
#15616=EDGE_LOOP('',(#69983,#69984,#69985,#69986));
#15617=EDGE_LOOP('',(#69987,#69988,#69989,#69990));
#15618=EDGE_LOOP('',(#69991,#69992,#69993,#69994));
#15619=EDGE_LOOP('',(#69995,#69996,#69997,#69998,#69999));
#15620=EDGE_LOOP('',(#70000,#70001,#70002,#70003));
#15621=EDGE_LOOP('',(#70004,#70005,#70006,#70007));
#15622=EDGE_LOOP('',(#70008,#70009,#70010,#70011));
#15623=EDGE_LOOP('',(#70012,#70013,#70014,#70015));
#15624=EDGE_LOOP('',(#70016,#70017,#70018,#70019));
#15625=EDGE_LOOP('',(#70020,#70021,#70022,#70023));
#15626=EDGE_LOOP('',(#70024,#70025,#70026,#70027));
#15627=EDGE_LOOP('',(#70028,#70029,#70030,#70031));
#15628=EDGE_LOOP('',(#70032,#70033,#70034,#70035,#70036));
#15629=EDGE_LOOP('',(#70037,#70038,#70039,#70040));
#15630=EDGE_LOOP('',(#70041,#70042,#70043,#70044));
#15631=EDGE_LOOP('',(#70045,#70046,#70047,#70048,#70049));
#15632=EDGE_LOOP('',(#70050,#70051,#70052,#70053));
#15633=EDGE_LOOP('',(#70054,#70055,#70056,#70057));
#15634=EDGE_LOOP('',(#70058,#70059,#70060,#70061));
#15635=EDGE_LOOP('',(#70062,#70063,#70064,#70065));
#15636=EDGE_LOOP('',(#70066,#70067,#70068,#70069,#70070));
#15637=EDGE_LOOP('',(#70071,#70072,#70073,#70074));
#15638=EDGE_LOOP('',(#70075,#70076,#70077,#70078));
#15639=EDGE_LOOP('',(#70079,#70080,#70081,#70082));
#15640=EDGE_LOOP('',(#70083,#70084,#70085,#70086));
#15641=EDGE_LOOP('',(#70087,#70088,#70089,#70090));
#15642=EDGE_LOOP('',(#70091,#70092,#70093,#70094));
#15643=EDGE_LOOP('',(#70095,#70096,#70097,#70098));
#15644=EDGE_LOOP('',(#70099,#70100,#70101,#70102));
#15645=EDGE_LOOP('',(#70103,#70104,#70105,#70106,#70107));
#15646=EDGE_LOOP('',(#70108,#70109,#70110,#70111));
#15647=EDGE_LOOP('',(#70112,#70113,#70114,#70115));
#15648=EDGE_LOOP('',(#70116,#70117,#70118,#70119));
#15649=EDGE_LOOP('',(#70120,#70121,#70122,#70123));
#15650=EDGE_LOOP('',(#70124,#70125,#70126,#70127));
#15651=EDGE_LOOP('',(#70128,#70129,#70130,#70131));
#15652=EDGE_LOOP('',(#70132,#70133,#70134,#70135));
#15653=EDGE_LOOP('',(#70136,#70137,#70138,#70139));
#15654=EDGE_LOOP('',(#70140,#70141,#70142,#70143,#70144));
#15655=EDGE_LOOP('',(#70145,#70146,#70147,#70148));
#15656=EDGE_LOOP('',(#70149,#70150,#70151,#70152));
#15657=EDGE_LOOP('',(#70153,#70154,#70155,#70156,#70157));
#15658=EDGE_LOOP('',(#70158,#70159,#70160,#70161));
#15659=EDGE_LOOP('',(#70162,#70163,#70164,#70165));
#15660=EDGE_LOOP('',(#70166,#70167,#70168,#70169));
#15661=EDGE_LOOP('',(#70170,#70171,#70172,#70173));
#15662=EDGE_LOOP('',(#70174,#70175,#70176,#70177,#70178));
#15663=EDGE_LOOP('',(#70179,#70180,#70181,#70182));
#15664=EDGE_LOOP('',(#70183,#70184,#70185,#70186));
#15665=EDGE_LOOP('',(#70187,#70188,#70189,#70190));
#15666=EDGE_LOOP('',(#70191,#70192,#70193,#70194));
#15667=EDGE_LOOP('',(#70195,#70196,#70197,#70198));
#15668=EDGE_LOOP('',(#70199,#70200,#70201,#70202));
#15669=EDGE_LOOP('',(#70203,#70204,#70205,#70206));
#15670=EDGE_LOOP('',(#70207,#70208,#70209,#70210));
#15671=EDGE_LOOP('',(#70211,#70212,#70213,#70214));
#15672=EDGE_LOOP('',(#70215,#70216,#70217,#70218));
#15673=EDGE_LOOP('',(#70219,#70220,#70221,#70222,#70223));
#15674=EDGE_LOOP('',(#70224,#70225,#70226,#70227));
#15675=EDGE_LOOP('',(#70228,#70229,#70230,#70231));
#15676=EDGE_LOOP('',(#70232,#70233,#70234,#70235));
#15677=EDGE_LOOP('',(#70236,#70237,#70238,#70239));
#15678=EDGE_LOOP('',(#70240,#70241,#70242,#70243));
#15679=EDGE_LOOP('',(#70244,#70245,#70246,#70247));
#15680=EDGE_LOOP('',(#70248,#70249,#70250,#70251));
#15681=EDGE_LOOP('',(#70252,#70253,#70254,#70255));
#15682=EDGE_LOOP('',(#70256,#70257,#70258,#70259,#70260));
#15683=EDGE_LOOP('',(#70261,#70262,#70263,#70264));
#15684=EDGE_LOOP('',(#70265,#70266,#70267,#70268));
#15685=EDGE_LOOP('',(#70269,#70270,#70271,#70272,#70273));
#15686=EDGE_LOOP('',(#70274,#70275,#70276,#70277));
#15687=EDGE_LOOP('',(#70278,#70279,#70280,#70281));
#15688=EDGE_LOOP('',(#70282,#70283,#70284,#70285));
#15689=EDGE_LOOP('',(#70286,#70287,#70288,#70289));
#15690=EDGE_LOOP('',(#70290,#70291,#70292,#70293,#70294));
#15691=EDGE_LOOP('',(#70295,#70296,#70297,#70298));
#15692=EDGE_LOOP('',(#70299,#70300,#70301,#70302));
#15693=EDGE_LOOP('',(#70303,#70304,#70305,#70306));
#15694=EDGE_LOOP('',(#70307,#70308,#70309,#70310));
#15695=EDGE_LOOP('',(#70311,#70312,#70313,#70314));
#15696=EDGE_LOOP('',(#70315,#70316,#70317,#70318));
#15697=EDGE_LOOP('',(#70319,#70320,#70321,#70322));
#15698=EDGE_LOOP('',(#70323,#70324,#70325,#70326));
#15699=EDGE_LOOP('',(#70327,#70328,#70329,#70330));
#15700=EDGE_LOOP('',(#70331,#70332,#70333,#70334));
#15701=EDGE_LOOP('',(#70335,#70336,#70337,#70338,#70339));
#15702=EDGE_LOOP('',(#70340,#70341,#70342,#70343));
#15703=EDGE_LOOP('',(#70344,#70345,#70346,#70347));
#15704=EDGE_LOOP('',(#70348,#70349,#70350,#70351));
#15705=EDGE_LOOP('',(#70352,#70353,#70354,#70355));
#15706=EDGE_LOOP('',(#70356,#70357,#70358,#70359));
#15707=EDGE_LOOP('',(#70360,#70361,#70362,#70363));
#15708=EDGE_LOOP('',(#70364,#70365,#70366,#70367));
#15709=EDGE_LOOP('',(#70368,#70369,#70370,#70371));
#15710=EDGE_LOOP('',(#70372,#70373,#70374,#70375,#70376));
#15711=EDGE_LOOP('',(#70377,#70378,#70379,#70380));
#15712=EDGE_LOOP('',(#70381,#70382,#70383,#70384));
#15713=EDGE_LOOP('',(#70385,#70386,#70387,#70388,#70389));
#15714=EDGE_LOOP('',(#70390,#70391,#70392,#70393));
#15715=EDGE_LOOP('',(#70394,#70395,#70396,#70397));
#15716=EDGE_LOOP('',(#70398,#70399,#70400,#70401));
#15717=EDGE_LOOP('',(#70402,#70403,#70404,#70405));
#15718=EDGE_LOOP('',(#70406,#70407,#70408,#70409,#70410));
#15719=EDGE_LOOP('',(#70411,#70412,#70413,#70414));
#15720=EDGE_LOOP('',(#70415,#70416,#70417,#70418));
#15721=EDGE_LOOP('',(#70419,#70420,#70421,#70422));
#15722=EDGE_LOOP('',(#70423,#70424,#70425,#70426));
#15723=EDGE_LOOP('',(#70427,#70428,#70429,#70430));
#15724=EDGE_LOOP('',(#70431,#70432,#70433,#70434));
#15725=EDGE_LOOP('',(#70435,#70436,#70437,#70438));
#15726=EDGE_LOOP('',(#70439,#70440,#70441,#70442));
#15727=EDGE_LOOP('',(#70443,#70444,#70445,#70446));
#15728=EDGE_LOOP('',(#70447,#70448,#70449,#70450));
#15729=EDGE_LOOP('',(#70451,#70452,#70453,#70454,#70455));
#15730=EDGE_LOOP('',(#70456,#70457,#70458,#70459));
#15731=EDGE_LOOP('',(#70460,#70461,#70462,#70463));
#15732=EDGE_LOOP('',(#70464,#70465,#70466,#70467));
#15733=EDGE_LOOP('',(#70468,#70469,#70470,#70471));
#15734=EDGE_LOOP('',(#70472,#70473,#70474,#70475));
#15735=EDGE_LOOP('',(#70476,#70477,#70478,#70479));
#15736=EDGE_LOOP('',(#70480,#70481,#70482,#70483));
#15737=EDGE_LOOP('',(#70484,#70485,#70486,#70487));
#15738=EDGE_LOOP('',(#70488,#70489,#70490,#70491,#70492));
#15739=EDGE_LOOP('',(#70493,#70494,#70495,#70496));
#15740=EDGE_LOOP('',(#70497,#70498,#70499,#70500));
#15741=EDGE_LOOP('',(#70501,#70502,#70503,#70504,#70505));
#15742=EDGE_LOOP('',(#70506,#70507,#70508,#70509));
#15743=EDGE_LOOP('',(#70510,#70511,#70512,#70513));
#15744=EDGE_LOOP('',(#70514,#70515,#70516,#70517));
#15745=EDGE_LOOP('',(#70518,#70519,#70520,#70521));
#15746=EDGE_LOOP('',(#70522,#70523,#70524,#70525,#70526));
#15747=EDGE_LOOP('',(#70527,#70528,#70529,#70530));
#15748=EDGE_LOOP('',(#70531,#70532,#70533,#70534));
#15749=EDGE_LOOP('',(#70535,#70536,#70537,#70538));
#15750=EDGE_LOOP('',(#70539,#70540,#70541,#70542));
#15751=EDGE_LOOP('',(#70543,#70544,#70545,#70546));
#15752=EDGE_LOOP('',(#70547,#70548,#70549,#70550));
#15753=EDGE_LOOP('',(#70551,#70552,#70553,#70554));
#15754=EDGE_LOOP('',(#70555,#70556,#70557,#70558));
#15755=EDGE_LOOP('',(#70559,#70560,#70561,#70562));
#15756=EDGE_LOOP('',(#70563,#70564,#70565,#70566));
#15757=EDGE_LOOP('',(#70567,#70568,#70569,#70570,#70571));
#15758=EDGE_LOOP('',(#70572,#70573,#70574,#70575));
#15759=EDGE_LOOP('',(#70576,#70577,#70578,#70579));
#15760=EDGE_LOOP('',(#70580,#70581,#70582,#70583));
#15761=EDGE_LOOP('',(#70584,#70585,#70586,#70587));
#15762=EDGE_LOOP('',(#70588,#70589,#70590,#70591));
#15763=EDGE_LOOP('',(#70592,#70593,#70594,#70595));
#15764=EDGE_LOOP('',(#70596,#70597,#70598,#70599));
#15765=EDGE_LOOP('',(#70600,#70601,#70602,#70603));
#15766=EDGE_LOOP('',(#70604,#70605,#70606,#70607,#70608));
#15767=EDGE_LOOP('',(#70609,#70610,#70611,#70612));
#15768=EDGE_LOOP('',(#70613,#70614,#70615,#70616));
#15769=EDGE_LOOP('',(#70617,#70618,#70619,#70620,#70621));
#15770=EDGE_LOOP('',(#70622,#70623,#70624,#70625));
#15771=EDGE_LOOP('',(#70626,#70627,#70628,#70629));
#15772=EDGE_LOOP('',(#70630,#70631,#70632,#70633));
#15773=EDGE_LOOP('',(#70634,#70635,#70636,#70637));
#15774=EDGE_LOOP('',(#70638,#70639,#70640,#70641,#70642));
#15775=EDGE_LOOP('',(#70643,#70644,#70645,#70646));
#15776=EDGE_LOOP('',(#70647,#70648,#70649,#70650));
#15777=EDGE_LOOP('',(#70651,#70652,#70653,#70654));
#15778=EDGE_LOOP('',(#70655,#70656,#70657,#70658));
#15779=EDGE_LOOP('',(#70659,#70660,#70661,#70662));
#15780=EDGE_LOOP('',(#70663,#70664,#70665,#70666));
#15781=EDGE_LOOP('',(#70667,#70668,#70669,#70670));
#15782=EDGE_LOOP('',(#70671,#70672,#70673,#70674));
#15783=EDGE_LOOP('',(#70675,#70676,#70677,#70678));
#15784=EDGE_LOOP('',(#70679,#70680,#70681,#70682));
#15785=EDGE_LOOP('',(#70683,#70684,#70685,#70686,#70687));
#15786=EDGE_LOOP('',(#70688,#70689,#70690,#70691));
#15787=EDGE_LOOP('',(#70692,#70693,#70694,#70695));
#15788=EDGE_LOOP('',(#70696,#70697,#70698,#70699));
#15789=EDGE_LOOP('',(#70700,#70701,#70702,#70703));
#15790=EDGE_LOOP('',(#70704,#70705,#70706,#70707));
#15791=EDGE_LOOP('',(#70708,#70709,#70710,#70711));
#15792=EDGE_LOOP('',(#70712,#70713,#70714,#70715));
#15793=EDGE_LOOP('',(#70716,#70717,#70718,#70719));
#15794=EDGE_LOOP('',(#70720,#70721,#70722,#70723,#70724));
#15795=EDGE_LOOP('',(#70725,#70726,#70727,#70728));
#15796=EDGE_LOOP('',(#70729,#70730,#70731,#70732));
#15797=EDGE_LOOP('',(#70733,#70734,#70735,#70736,#70737));
#15798=EDGE_LOOP('',(#70738,#70739,#70740,#70741));
#15799=EDGE_LOOP('',(#70742,#70743,#70744,#70745));
#15800=EDGE_LOOP('',(#70746,#70747,#70748,#70749));
#15801=EDGE_LOOP('',(#70750,#70751,#70752,#70753));
#15802=EDGE_LOOP('',(#70754,#70755,#70756,#70757,#70758));
#15803=EDGE_LOOP('',(#70759,#70760,#70761,#70762));
#15804=EDGE_LOOP('',(#70763,#70764,#70765,#70766));
#15805=EDGE_LOOP('',(#70767,#70768,#70769,#70770));
#15806=EDGE_LOOP('',(#70771,#70772,#70773,#70774));
#15807=EDGE_LOOP('',(#70775,#70776,#70777,#70778));
#15808=EDGE_LOOP('',(#70779,#70780,#70781,#70782));
#15809=EDGE_LOOP('',(#70783,#70784,#70785,#70786));
#15810=EDGE_LOOP('',(#70787,#70788,#70789,#70790));
#15811=EDGE_LOOP('',(#70791,#70792,#70793,#70794));
#15812=EDGE_LOOP('',(#70795,#70796,#70797,#70798));
#15813=EDGE_LOOP('',(#70799,#70800,#70801,#70802,#70803));
#15814=EDGE_LOOP('',(#70804,#70805,#70806,#70807));
#15815=EDGE_LOOP('',(#70808,#70809,#70810,#70811));
#15816=EDGE_LOOP('',(#70812,#70813,#70814,#70815));
#15817=EDGE_LOOP('',(#70816,#70817,#70818,#70819));
#15818=EDGE_LOOP('',(#70820,#70821,#70822,#70823));
#15819=EDGE_LOOP('',(#70824,#70825,#70826,#70827));
#15820=EDGE_LOOP('',(#70828,#70829,#70830,#70831));
#15821=EDGE_LOOP('',(#70832,#70833,#70834,#70835));
#15822=EDGE_LOOP('',(#70836,#70837,#70838,#70839,#70840));
#15823=EDGE_LOOP('',(#70841,#70842,#70843,#70844));
#15824=EDGE_LOOP('',(#70845,#70846,#70847,#70848));
#15825=EDGE_LOOP('',(#70849,#70850,#70851,#70852,#70853));
#15826=EDGE_LOOP('',(#70854,#70855,#70856,#70857));
#15827=EDGE_LOOP('',(#70858,#70859,#70860,#70861));
#15828=EDGE_LOOP('',(#70862,#70863,#70864,#70865));
#15829=EDGE_LOOP('',(#70866,#70867,#70868,#70869));
#15830=EDGE_LOOP('',(#70870,#70871,#70872,#70873,#70874));
#15831=EDGE_LOOP('',(#70875,#70876,#70877,#70878));
#15832=EDGE_LOOP('',(#70879,#70880,#70881,#70882));
#15833=EDGE_LOOP('',(#70883,#70884,#70885,#70886));
#15834=EDGE_LOOP('',(#70887,#70888,#70889,#70890));
#15835=EDGE_LOOP('',(#70891,#70892,#70893,#70894));
#15836=EDGE_LOOP('',(#70895,#70896,#70897,#70898));
#15837=EDGE_LOOP('',(#70899,#70900,#70901,#70902));
#15838=EDGE_LOOP('',(#70903,#70904,#70905,#70906));
#15839=EDGE_LOOP('',(#70907,#70908,#70909,#70910));
#15840=EDGE_LOOP('',(#70911,#70912,#70913,#70914));
#15841=EDGE_LOOP('',(#70915,#70916,#70917,#70918,#70919));
#15842=EDGE_LOOP('',(#70920,#70921,#70922,#70923));
#15843=EDGE_LOOP('',(#70924,#70925,#70926,#70927));
#15844=EDGE_LOOP('',(#70928,#70929,#70930,#70931));
#15845=EDGE_LOOP('',(#70932,#70933,#70934,#70935));
#15846=EDGE_LOOP('',(#70936,#70937,#70938,#70939));
#15847=EDGE_LOOP('',(#70940,#70941,#70942,#70943));
#15848=EDGE_LOOP('',(#70944,#70945,#70946,#70947));
#15849=EDGE_LOOP('',(#70948,#70949,#70950,#70951));
#15850=EDGE_LOOP('',(#70952,#70953,#70954,#70955,#70956));
#15851=EDGE_LOOP('',(#70957,#70958,#70959,#70960));
#15852=EDGE_LOOP('',(#70961,#70962,#70963,#70964));
#15853=EDGE_LOOP('',(#70965,#70966,#70967,#70968,#70969));
#15854=EDGE_LOOP('',(#70970,#70971,#70972,#70973));
#15855=EDGE_LOOP('',(#70974,#70975,#70976,#70977));
#15856=EDGE_LOOP('',(#70978,#70979,#70980,#70981));
#15857=EDGE_LOOP('',(#70982,#70983,#70984,#70985));
#15858=EDGE_LOOP('',(#70986,#70987,#70988,#70989,#70990));
#15859=EDGE_LOOP('',(#70991,#70992,#70993,#70994));
#15860=EDGE_LOOP('',(#70995,#70996,#70997,#70998));
#15861=EDGE_LOOP('',(#70999,#71000,#71001,#71002));
#15862=EDGE_LOOP('',(#71003,#71004,#71005,#71006));
#15863=EDGE_LOOP('',(#71007,#71008,#71009,#71010));
#15864=EDGE_LOOP('',(#71011,#71012,#71013,#71014));
#15865=EDGE_LOOP('',(#71015,#71016,#71017,#71018));
#15866=EDGE_LOOP('',(#71019,#71020,#71021,#71022));
#15867=EDGE_LOOP('',(#71023,#71024,#71025,#71026));
#15868=EDGE_LOOP('',(#71027,#71028,#71029,#71030));
#15869=EDGE_LOOP('',(#71031,#71032,#71033,#71034,#71035));
#15870=EDGE_LOOP('',(#71036,#71037,#71038,#71039));
#15871=EDGE_LOOP('',(#71040,#71041,#71042,#71043));
#15872=EDGE_LOOP('',(#71044,#71045,#71046,#71047));
#15873=EDGE_LOOP('',(#71048,#71049,#71050,#71051));
#15874=EDGE_LOOP('',(#71052,#71053,#71054,#71055));
#15875=EDGE_LOOP('',(#71056,#71057,#71058,#71059));
#15876=EDGE_LOOP('',(#71060,#71061,#71062,#71063));
#15877=EDGE_LOOP('',(#71064,#71065,#71066,#71067));
#15878=EDGE_LOOP('',(#71068,#71069,#71070,#71071,#71072));
#15879=EDGE_LOOP('',(#71073,#71074,#71075,#71076));
#15880=EDGE_LOOP('',(#71077,#71078,#71079,#71080));
#15881=EDGE_LOOP('',(#71081,#71082,#71083,#71084,#71085));
#15882=EDGE_LOOP('',(#71086,#71087,#71088,#71089));
#15883=EDGE_LOOP('',(#71090,#71091,#71092,#71093));
#15884=EDGE_LOOP('',(#71094,#71095,#71096,#71097));
#15885=EDGE_LOOP('',(#71098,#71099,#71100,#71101));
#15886=EDGE_LOOP('',(#71102,#71103,#71104,#71105,#71106));
#15887=EDGE_LOOP('',(#71107,#71108,#71109,#71110));
#15888=EDGE_LOOP('',(#71111,#71112,#71113,#71114));
#15889=EDGE_LOOP('',(#71115,#71116,#71117,#71118));
#15890=EDGE_LOOP('',(#71119,#71120,#71121,#71122));
#15891=EDGE_LOOP('',(#71123,#71124,#71125,#71126));
#15892=EDGE_LOOP('',(#71127,#71128,#71129,#71130));
#15893=EDGE_LOOP('',(#71131,#71132,#71133,#71134));
#15894=EDGE_LOOP('',(#71135,#71136,#71137,#71138));
#15895=EDGE_LOOP('',(#71139,#71140,#71141,#71142));
#15896=EDGE_LOOP('',(#71143,#71144,#71145,#71146));
#15897=EDGE_LOOP('',(#71147,#71148,#71149,#71150,#71151));
#15898=EDGE_LOOP('',(#71152,#71153,#71154,#71155));
#15899=EDGE_LOOP('',(#71156,#71157,#71158,#71159));
#15900=EDGE_LOOP('',(#71160,#71161,#71162,#71163));
#15901=EDGE_LOOP('',(#71164,#71165,#71166,#71167));
#15902=EDGE_LOOP('',(#71168,#71169,#71170,#71171));
#15903=EDGE_LOOP('',(#71172,#71173,#71174,#71175));
#15904=EDGE_LOOP('',(#71176,#71177,#71178,#71179));
#15905=EDGE_LOOP('',(#71180,#71181,#71182,#71183));
#15906=EDGE_LOOP('',(#71184,#71185,#71186,#71187,#71188));
#15907=EDGE_LOOP('',(#71189,#71190,#71191,#71192));
#15908=EDGE_LOOP('',(#71193,#71194,#71195,#71196));
#15909=EDGE_LOOP('',(#71197,#71198,#71199,#71200,#71201));
#15910=EDGE_LOOP('',(#71202,#71203,#71204,#71205));
#15911=EDGE_LOOP('',(#71206,#71207,#71208,#71209));
#15912=EDGE_LOOP('',(#71210,#71211,#71212,#71213));
#15913=EDGE_LOOP('',(#71214,#71215,#71216,#71217));
#15914=EDGE_LOOP('',(#71218,#71219,#71220,#71221,#71222));
#15915=EDGE_LOOP('',(#71223,#71224,#71225,#71226));
#15916=EDGE_LOOP('',(#71227,#71228,#71229,#71230));
#15917=EDGE_LOOP('',(#71231,#71232,#71233,#71234));
#15918=EDGE_LOOP('',(#71235,#71236,#71237,#71238));
#15919=EDGE_LOOP('',(#71239,#71240,#71241,#71242));
#15920=EDGE_LOOP('',(#71243,#71244,#71245,#71246));
#15921=EDGE_LOOP('',(#71247,#71248,#71249,#71250));
#15922=EDGE_LOOP('',(#71251,#71252,#71253,#71254));
#15923=EDGE_LOOP('',(#71255,#71256,#71257,#71258));
#15924=EDGE_LOOP('',(#71259,#71260,#71261,#71262));
#15925=EDGE_LOOP('',(#71263,#71264,#71265,#71266,#71267));
#15926=EDGE_LOOP('',(#71268,#71269,#71270,#71271));
#15927=EDGE_LOOP('',(#71272,#71273,#71274,#71275));
#15928=EDGE_LOOP('',(#71276,#71277,#71278,#71279));
#15929=EDGE_LOOP('',(#71280,#71281,#71282,#71283));
#15930=EDGE_LOOP('',(#71284,#71285,#71286,#71287));
#15931=EDGE_LOOP('',(#71288,#71289,#71290,#71291));
#15932=EDGE_LOOP('',(#71292,#71293,#71294,#71295));
#15933=EDGE_LOOP('',(#71296,#71297,#71298,#71299));
#15934=EDGE_LOOP('',(#71300,#71301,#71302,#71303,#71304));
#15935=EDGE_LOOP('',(#71305,#71306,#71307,#71308));
#15936=EDGE_LOOP('',(#71309,#71310,#71311,#71312));
#15937=EDGE_LOOP('',(#71313,#71314,#71315,#71316,#71317));
#15938=EDGE_LOOP('',(#71318,#71319,#71320,#71321));
#15939=EDGE_LOOP('',(#71322,#71323,#71324,#71325));
#15940=EDGE_LOOP('',(#71326,#71327,#71328,#71329));
#15941=EDGE_LOOP('',(#71330,#71331,#71332,#71333));
#15942=EDGE_LOOP('',(#71334,#71335,#71336,#71337,#71338));
#15943=EDGE_LOOP('',(#71339,#71340,#71341,#71342));
#15944=EDGE_LOOP('',(#71343,#71344,#71345,#71346));
#15945=EDGE_LOOP('',(#71347,#71348,#71349,#71350));
#15946=EDGE_LOOP('',(#71351,#71352,#71353,#71354));
#15947=EDGE_LOOP('',(#71355,#71356,#71357,#71358));
#15948=EDGE_LOOP('',(#71359,#71360,#71361,#71362));
#15949=EDGE_LOOP('',(#71363,#71364,#71365,#71366));
#15950=EDGE_LOOP('',(#71367,#71368,#71369,#71370));
#15951=EDGE_LOOP('',(#71371,#71372,#71373,#71374));
#15952=EDGE_LOOP('',(#71375,#71376,#71377,#71378));
#15953=EDGE_LOOP('',(#71379,#71380,#71381,#71382,#71383));
#15954=EDGE_LOOP('',(#71384,#71385,#71386,#71387));
#15955=EDGE_LOOP('',(#71388,#71389,#71390,#71391));
#15956=EDGE_LOOP('',(#71392,#71393,#71394,#71395));
#15957=EDGE_LOOP('',(#71396,#71397,#71398,#71399));
#15958=EDGE_LOOP('',(#71400,#71401,#71402,#71403));
#15959=EDGE_LOOP('',(#71404,#71405,#71406,#71407));
#15960=EDGE_LOOP('',(#71408,#71409,#71410,#71411));
#15961=EDGE_LOOP('',(#71412,#71413,#71414,#71415));
#15962=EDGE_LOOP('',(#71416,#71417,#71418,#71419,#71420));
#15963=EDGE_LOOP('',(#71421,#71422,#71423,#71424));
#15964=EDGE_LOOP('',(#71425,#71426,#71427,#71428));
#15965=EDGE_LOOP('',(#71429,#71430,#71431,#71432,#71433));
#15966=EDGE_LOOP('',(#71434,#71435,#71436,#71437));
#15967=EDGE_LOOP('',(#71438,#71439,#71440,#71441));
#15968=EDGE_LOOP('',(#71442,#71443,#71444,#71445));
#15969=EDGE_LOOP('',(#71446,#71447,#71448,#71449));
#15970=EDGE_LOOP('',(#71450,#71451,#71452,#71453,#71454));
#15971=EDGE_LOOP('',(#71455,#71456,#71457,#71458));
#15972=EDGE_LOOP('',(#71459,#71460,#71461,#71462));
#15973=EDGE_LOOP('',(#71463,#71464,#71465,#71466));
#15974=EDGE_LOOP('',(#71467,#71468,#71469,#71470));
#15975=EDGE_LOOP('',(#71471,#71472,#71473,#71474));
#15976=EDGE_LOOP('',(#71475,#71476,#71477,#71478));
#15977=EDGE_LOOP('',(#71479,#71480,#71481,#71482));
#15978=EDGE_LOOP('',(#71483,#71484,#71485,#71486));
#15979=EDGE_LOOP('',(#71487,#71488,#71489,#71490));
#15980=EDGE_LOOP('',(#71491,#71492,#71493,#71494));
#15981=EDGE_LOOP('',(#71495,#71496,#71497,#71498,#71499));
#15982=EDGE_LOOP('',(#71500,#71501,#71502,#71503));
#15983=EDGE_LOOP('',(#71504,#71505,#71506,#71507));
#15984=EDGE_LOOP('',(#71508,#71509,#71510,#71511));
#15985=EDGE_LOOP('',(#71512,#71513,#71514,#71515));
#15986=EDGE_LOOP('',(#71516,#71517,#71518,#71519));
#15987=EDGE_LOOP('',(#71520,#71521,#71522,#71523));
#15988=EDGE_LOOP('',(#71524,#71525,#71526,#71527));
#15989=EDGE_LOOP('',(#71528,#71529,#71530,#71531));
#15990=EDGE_LOOP('',(#71532,#71533,#71534,#71535,#71536));
#15991=EDGE_LOOP('',(#71537,#71538,#71539,#71540));
#15992=EDGE_LOOP('',(#71541,#71542,#71543,#71544));
#15993=EDGE_LOOP('',(#71545,#71546,#71547,#71548,#71549));
#15994=EDGE_LOOP('',(#71550,#71551,#71552,#71553));
#15995=EDGE_LOOP('',(#71554,#71555,#71556,#71557));
#15996=EDGE_LOOP('',(#71558,#71559,#71560,#71561));
#15997=EDGE_LOOP('',(#71562,#71563,#71564,#71565));
#15998=EDGE_LOOP('',(#71566,#71567,#71568,#71569,#71570));
#15999=EDGE_LOOP('',(#71571,#71572,#71573,#71574));
#16000=EDGE_LOOP('',(#71575,#71576,#71577,#71578));
#16001=EDGE_LOOP('',(#71579,#71580,#71581,#71582));
#16002=EDGE_LOOP('',(#71583,#71584,#71585,#71586));
#16003=EDGE_LOOP('',(#71587,#71588,#71589,#71590));
#16004=EDGE_LOOP('',(#71591,#71592,#71593,#71594));
#16005=EDGE_LOOP('',(#71595,#71596,#71597,#71598));
#16006=EDGE_LOOP('',(#71599,#71600,#71601,#71602));
#16007=EDGE_LOOP('',(#71603,#71604,#71605,#71606));
#16008=EDGE_LOOP('',(#71607,#71608,#71609,#71610));
#16009=EDGE_LOOP('',(#71611,#71612,#71613,#71614,#71615));
#16010=EDGE_LOOP('',(#71616,#71617,#71618,#71619));
#16011=EDGE_LOOP('',(#71620,#71621,#71622,#71623));
#16012=EDGE_LOOP('',(#71624,#71625,#71626,#71627));
#16013=EDGE_LOOP('',(#71628,#71629,#71630,#71631));
#16014=EDGE_LOOP('',(#71632,#71633,#71634,#71635));
#16015=EDGE_LOOP('',(#71636,#71637,#71638,#71639));
#16016=EDGE_LOOP('',(#71640,#71641,#71642,#71643));
#16017=EDGE_LOOP('',(#71644,#71645,#71646,#71647));
#16018=EDGE_LOOP('',(#71648,#71649,#71650,#71651,#71652));
#16019=EDGE_LOOP('',(#71653,#71654,#71655,#71656));
#16020=EDGE_LOOP('',(#71657,#71658,#71659,#71660));
#16021=EDGE_LOOP('',(#71661,#71662,#71663,#71664,#71665));
#16022=EDGE_LOOP('',(#71666,#71667,#71668,#71669));
#16023=EDGE_LOOP('',(#71670,#71671,#71672,#71673));
#16024=EDGE_LOOP('',(#71674,#71675,#71676,#71677));
#16025=EDGE_LOOP('',(#71678,#71679,#71680,#71681));
#16026=EDGE_LOOP('',(#71682,#71683,#71684,#71685,#71686));
#16027=EDGE_LOOP('',(#71687,#71688,#71689,#71690));
#16028=EDGE_LOOP('',(#71691,#71692,#71693,#71694));
#16029=EDGE_LOOP('',(#71695,#71696,#71697,#71698));
#16030=EDGE_LOOP('',(#71699,#71700,#71701,#71702));
#16031=EDGE_LOOP('',(#71703,#71704,#71705,#71706));
#16032=EDGE_LOOP('',(#71707,#71708,#71709,#71710));
#16033=EDGE_LOOP('',(#71711,#71712,#71713,#71714));
#16034=EDGE_LOOP('',(#71715,#71716,#71717,#71718));
#16035=EDGE_LOOP('',(#71719,#71720,#71721,#71722));
#16036=EDGE_LOOP('',(#71723,#71724,#71725,#71726));
#16037=EDGE_LOOP('',(#71727,#71728,#71729,#71730,#71731));
#16038=EDGE_LOOP('',(#71732,#71733,#71734,#71735));
#16039=EDGE_LOOP('',(#71736,#71737,#71738,#71739));
#16040=EDGE_LOOP('',(#71740,#71741,#71742,#71743));
#16041=EDGE_LOOP('',(#71744,#71745,#71746,#71747));
#16042=EDGE_LOOP('',(#71748,#71749,#71750,#71751));
#16043=EDGE_LOOP('',(#71752,#71753,#71754,#71755));
#16044=EDGE_LOOP('',(#71756,#71757,#71758,#71759));
#16045=EDGE_LOOP('',(#71760,#71761,#71762,#71763));
#16046=EDGE_LOOP('',(#71764,#71765,#71766,#71767,#71768));
#16047=EDGE_LOOP('',(#71769,#71770,#71771,#71772));
#16048=EDGE_LOOP('',(#71773,#71774,#71775,#71776));
#16049=EDGE_LOOP('',(#71777,#71778,#71779,#71780,#71781));
#16050=EDGE_LOOP('',(#71782,#71783,#71784,#71785));
#16051=EDGE_LOOP('',(#71786,#71787,#71788,#71789));
#16052=EDGE_LOOP('',(#71790,#71791,#71792,#71793));
#16053=EDGE_LOOP('',(#71794,#71795,#71796,#71797));
#16054=EDGE_LOOP('',(#71798,#71799,#71800,#71801,#71802));
#16055=EDGE_LOOP('',(#71803,#71804,#71805,#71806));
#16056=EDGE_LOOP('',(#71807,#71808,#71809,#71810));
#16057=EDGE_LOOP('',(#71811,#71812,#71813,#71814));
#16058=EDGE_LOOP('',(#71815,#71816,#71817,#71818));
#16059=EDGE_LOOP('',(#71819,#71820,#71821,#71822));
#16060=EDGE_LOOP('',(#71823,#71824,#71825,#71826));
#16061=EDGE_LOOP('',(#71827,#71828,#71829,#71830));
#16062=EDGE_LOOP('',(#71831,#71832,#71833,#71834));
#16063=EDGE_LOOP('',(#71835,#71836,#71837,#71838,#71839));
#16064=EDGE_LOOP('',(#71840,#71841,#71842,#71843));
#16065=EDGE_LOOP('',(#71844,#71845,#71846,#71847));
#16066=EDGE_LOOP('',(#71848,#71849,#71850,#71851));
#16067=EDGE_LOOP('',(#71852,#71853,#71854,#71855));
#16068=EDGE_LOOP('',(#71856,#71857,#71858,#71859));
#16069=EDGE_LOOP('',(#71860,#71861,#71862,#71863));
#16070=EDGE_LOOP('',(#71864,#71865,#71866,#71867));
#16071=EDGE_LOOP('',(#71868,#71869,#71870,#71871));
#16072=EDGE_LOOP('',(#71872,#71873,#71874,#71875,#71876));
#16073=EDGE_LOOP('',(#71877,#71878,#71879,#71880));
#16074=EDGE_LOOP('',(#71881,#71882,#71883,#71884));
#16075=EDGE_LOOP('',(#71885,#71886,#71887,#71888,#71889));
#16076=EDGE_LOOP('',(#71890,#71891,#71892,#71893));
#16077=EDGE_LOOP('',(#71894,#71895,#71896,#71897));
#16078=EDGE_LOOP('',(#71898,#71899,#71900,#71901));
#16079=EDGE_LOOP('',(#71902,#71903,#71904,#71905));
#16080=EDGE_LOOP('',(#71906,#71907,#71908,#71909,#71910));
#16081=EDGE_LOOP('',(#71911,#71912,#71913,#71914));
#16082=EDGE_LOOP('',(#71915,#71916,#71917,#71918));
#16083=EDGE_LOOP('',(#71919,#71920,#71921,#71922));
#16084=EDGE_LOOP('',(#71923,#71924,#71925,#71926));
#16085=EDGE_LOOP('',(#71927,#71928,#71929,#71930));
#16086=EDGE_LOOP('',(#71931,#71932,#71933,#71934));
#16087=EDGE_LOOP('',(#71935,#71936,#71937,#71938));
#16088=EDGE_LOOP('',(#71939,#71940,#71941,#71942));
#16089=EDGE_LOOP('',(#71943,#71944,#71945,#71946));
#16090=EDGE_LOOP('',(#71947,#71948,#71949,#71950));
#16091=EDGE_LOOP('',(#71951,#71952,#71953,#71954,#71955));
#16092=EDGE_LOOP('',(#71956,#71957,#71958,#71959));
#16093=EDGE_LOOP('',(#71960,#71961,#71962,#71963));
#16094=EDGE_LOOP('',(#71964,#71965,#71966,#71967));
#16095=EDGE_LOOP('',(#71968,#71969,#71970,#71971));
#16096=EDGE_LOOP('',(#71972,#71973,#71974,#71975));
#16097=EDGE_LOOP('',(#71976,#71977,#71978,#71979));
#16098=EDGE_LOOP('',(#71980,#71981,#71982,#71983));
#16099=EDGE_LOOP('',(#71984,#71985,#71986,#71987));
#16100=EDGE_LOOP('',(#71988,#71989,#71990,#71991,#71992));
#16101=EDGE_LOOP('',(#71993,#71994,#71995,#71996));
#16102=EDGE_LOOP('',(#71997,#71998,#71999,#72000));
#16103=EDGE_LOOP('',(#72001,#72002,#72003,#72004,#72005));
#16104=EDGE_LOOP('',(#72006,#72007,#72008,#72009));
#16105=EDGE_LOOP('',(#72010,#72011,#72012,#72013));
#16106=EDGE_LOOP('',(#72014,#72015,#72016,#72017));
#16107=EDGE_LOOP('',(#72018,#72019,#72020,#72021));
#16108=EDGE_LOOP('',(#72022,#72023,#72024,#72025,#72026));
#16109=EDGE_LOOP('',(#72027,#72028,#72029,#72030));
#16110=EDGE_LOOP('',(#72031,#72032,#72033,#72034));
#16111=EDGE_LOOP('',(#72035,#72036,#72037,#72038));
#16112=EDGE_LOOP('',(#72039,#72040,#72041,#72042));
#16113=EDGE_LOOP('',(#72043,#72044,#72045,#72046));
#16114=EDGE_LOOP('',(#72047,#72048,#72049,#72050));
#16115=EDGE_LOOP('',(#72051,#72052,#72053,#72054));
#16116=EDGE_LOOP('',(#72055,#72056,#72057,#72058));
#16117=EDGE_LOOP('',(#72059,#72060,#72061,#72062));
#16118=EDGE_LOOP('',(#72063,#72064,#72065,#72066));
#16119=EDGE_LOOP('',(#72067,#72068,#72069,#72070,#72071));
#16120=EDGE_LOOP('',(#72072,#72073,#72074,#72075));
#16121=EDGE_LOOP('',(#72076,#72077,#72078,#72079));
#16122=EDGE_LOOP('',(#72080,#72081,#72082,#72083));
#16123=EDGE_LOOP('',(#72084,#72085,#72086,#72087));
#16124=EDGE_LOOP('',(#72088,#72089,#72090,#72091));
#16125=EDGE_LOOP('',(#72092,#72093,#72094,#72095));
#16126=EDGE_LOOP('',(#72096,#72097,#72098,#72099));
#16127=EDGE_LOOP('',(#72100,#72101,#72102,#72103));
#16128=EDGE_LOOP('',(#72104,#72105,#72106,#72107,#72108));
#16129=EDGE_LOOP('',(#72109,#72110,#72111,#72112));
#16130=EDGE_LOOP('',(#72113,#72114,#72115,#72116));
#16131=EDGE_LOOP('',(#72117,#72118,#72119,#72120,#72121));
#16132=EDGE_LOOP('',(#72122,#72123,#72124,#72125));
#16133=EDGE_LOOP('',(#72126,#72127,#72128,#72129));
#16134=EDGE_LOOP('',(#72130,#72131,#72132,#72133));
#16135=EDGE_LOOP('',(#72134,#72135,#72136,#72137));
#16136=EDGE_LOOP('',(#72138,#72139,#72140,#72141,#72142));
#16137=EDGE_LOOP('',(#72143,#72144,#72145,#72146));
#16138=EDGE_LOOP('',(#72147,#72148,#72149,#72150));
#16139=EDGE_LOOP('',(#72151,#72152,#72153,#72154));
#16140=EDGE_LOOP('',(#72155,#72156,#72157,#72158));
#16141=EDGE_LOOP('',(#72159,#72160,#72161,#72162));
#16142=EDGE_LOOP('',(#72163,#72164,#72165,#72166));
#16143=EDGE_LOOP('',(#72167,#72168,#72169,#72170));
#16144=EDGE_LOOP('',(#72171,#72172,#72173,#72174));
#16145=EDGE_LOOP('',(#72175,#72176,#72177,#72178));
#16146=EDGE_LOOP('',(#72179,#72180,#72181,#72182));
#16147=EDGE_LOOP('',(#72183,#72184,#72185,#72186,#72187));
#16148=EDGE_LOOP('',(#72188,#72189,#72190,#72191));
#16149=EDGE_LOOP('',(#72192,#72193,#72194,#72195));
#16150=EDGE_LOOP('',(#72196,#72197,#72198,#72199));
#16151=EDGE_LOOP('',(#72200,#72201,#72202,#72203));
#16152=EDGE_LOOP('',(#72204,#72205,#72206,#72207));
#16153=EDGE_LOOP('',(#72208,#72209,#72210,#72211));
#16154=EDGE_LOOP('',(#72212,#72213,#72214,#72215));
#16155=EDGE_LOOP('',(#72216,#72217,#72218,#72219));
#16156=EDGE_LOOP('',(#72220,#72221,#72222,#72223,#72224));
#16157=EDGE_LOOP('',(#72225,#72226,#72227,#72228));
#16158=EDGE_LOOP('',(#72229,#72230,#72231,#72232));
#16159=EDGE_LOOP('',(#72233,#72234,#72235,#72236,#72237));
#16160=EDGE_LOOP('',(#72238,#72239,#72240,#72241));
#16161=EDGE_LOOP('',(#72242,#72243,#72244,#72245));
#16162=EDGE_LOOP('',(#72246,#72247,#72248,#72249));
#16163=EDGE_LOOP('',(#72250,#72251,#72252,#72253));
#16164=EDGE_LOOP('',(#72254,#72255,#72256,#72257,#72258));
#16165=EDGE_LOOP('',(#72259,#72260,#72261,#72262));
#16166=EDGE_LOOP('',(#72263,#72264,#72265,#72266));
#16167=EDGE_LOOP('',(#72267,#72268,#72269,#72270));
#16168=EDGE_LOOP('',(#72271,#72272,#72273,#72274));
#16169=EDGE_LOOP('',(#72275,#72276,#72277,#72278));
#16170=EDGE_LOOP('',(#72279,#72280,#72281,#72282));
#16171=EDGE_LOOP('',(#72283,#72284,#72285,#72286));
#16172=EDGE_LOOP('',(#72287,#72288,#72289,#72290));
#16173=EDGE_LOOP('',(#72291,#72292,#72293,#72294));
#16174=EDGE_LOOP('',(#72295,#72296,#72297,#72298));
#16175=EDGE_LOOP('',(#72299,#72300,#72301,#72302,#72303));
#16176=EDGE_LOOP('',(#72304,#72305,#72306,#72307));
#16177=EDGE_LOOP('',(#72308,#72309,#72310,#72311));
#16178=EDGE_LOOP('',(#72312,#72313,#72314,#72315));
#16179=EDGE_LOOP('',(#72316,#72317,#72318,#72319));
#16180=EDGE_LOOP('',(#72320,#72321,#72322,#72323));
#16181=EDGE_LOOP('',(#72324,#72325,#72326,#72327));
#16182=EDGE_LOOP('',(#72328,#72329,#72330,#72331));
#16183=EDGE_LOOP('',(#72332,#72333,#72334,#72335));
#16184=EDGE_LOOP('',(#72336,#72337,#72338,#72339,#72340));
#16185=EDGE_LOOP('',(#72341,#72342,#72343,#72344));
#16186=EDGE_LOOP('',(#72345,#72346,#72347,#72348));
#16187=EDGE_LOOP('',(#72349,#72350,#72351,#72352,#72353));
#16188=EDGE_LOOP('',(#72354,#72355,#72356,#72357));
#16189=EDGE_LOOP('',(#72358,#72359,#72360,#72361));
#16190=EDGE_LOOP('',(#72362,#72363,#72364,#72365));
#16191=EDGE_LOOP('',(#72366,#72367,#72368,#72369));
#16192=EDGE_LOOP('',(#72370,#72371,#72372,#72373,#72374));
#16193=EDGE_LOOP('',(#72375,#72376,#72377,#72378));
#16194=EDGE_LOOP('',(#72379,#72380,#72381,#72382));
#16195=EDGE_LOOP('',(#72383,#72384,#72385,#72386));
#16196=EDGE_LOOP('',(#72387,#72388,#72389,#72390));
#16197=EDGE_LOOP('',(#72391,#72392,#72393,#72394));
#16198=EDGE_LOOP('',(#72395,#72396,#72397,#72398));
#16199=EDGE_LOOP('',(#72399,#72400,#72401,#72402));
#16200=EDGE_LOOP('',(#72403,#72404,#72405,#72406));
#16201=EDGE_LOOP('',(#72407,#72408,#72409,#72410));
#16202=EDGE_LOOP('',(#72411,#72412,#72413,#72414));
#16203=EDGE_LOOP('',(#72415,#72416,#72417,#72418,#72419));
#16204=EDGE_LOOP('',(#72420,#72421,#72422,#72423));
#16205=EDGE_LOOP('',(#72424,#72425,#72426,#72427));
#16206=EDGE_LOOP('',(#72428,#72429,#72430,#72431));
#16207=EDGE_LOOP('',(#72432,#72433,#72434,#72435));
#16208=EDGE_LOOP('',(#72436,#72437,#72438,#72439));
#16209=EDGE_LOOP('',(#72440,#72441,#72442,#72443));
#16210=EDGE_LOOP('',(#72444,#72445,#72446,#72447));
#16211=EDGE_LOOP('',(#72448,#72449,#72450,#72451));
#16212=EDGE_LOOP('',(#72452,#72453,#72454,#72455,#72456));
#16213=EDGE_LOOP('',(#72457,#72458,#72459,#72460));
#16214=EDGE_LOOP('',(#72461,#72462,#72463,#72464));
#16215=EDGE_LOOP('',(#72465,#72466,#72467,#72468,#72469));
#16216=EDGE_LOOP('',(#72470,#72471,#72472,#72473));
#16217=EDGE_LOOP('',(#72474,#72475,#72476,#72477));
#16218=EDGE_LOOP('',(#72478,#72479,#72480,#72481));
#16219=EDGE_LOOP('',(#72482,#72483,#72484,#72485));
#16220=EDGE_LOOP('',(#72486,#72487,#72488,#72489,#72490));
#16221=EDGE_LOOP('',(#72491,#72492,#72493,#72494));
#16222=EDGE_LOOP('',(#72495,#72496,#72497,#72498));
#16223=EDGE_LOOP('',(#72499,#72500,#72501,#72502));
#16224=EDGE_LOOP('',(#72503,#72504,#72505,#72506));
#16225=EDGE_LOOP('',(#72507,#72508,#72509,#72510));
#16226=EDGE_LOOP('',(#72511,#72512,#72513,#72514));
#16227=EDGE_LOOP('',(#72515,#72516,#72517,#72518));
#16228=EDGE_LOOP('',(#72519,#72520,#72521,#72522));
#16229=EDGE_LOOP('',(#72523,#72524,#72525,#72526));
#16230=EDGE_LOOP('',(#72527,#72528,#72529,#72530));
#16231=EDGE_LOOP('',(#72531,#72532,#72533,#72534,#72535));
#16232=EDGE_LOOP('',(#72536,#72537,#72538,#72539));
#16233=EDGE_LOOP('',(#72540,#72541,#72542,#72543));
#16234=EDGE_LOOP('',(#72544,#72545,#72546,#72547));
#16235=EDGE_LOOP('',(#72548,#72549,#72550,#72551));
#16236=EDGE_LOOP('',(#72552,#72553,#72554,#72555));
#16237=EDGE_LOOP('',(#72556,#72557,#72558,#72559));
#16238=EDGE_LOOP('',(#72560,#72561,#72562,#72563));
#16239=EDGE_LOOP('',(#72564,#72565,#72566,#72567));
#16240=EDGE_LOOP('',(#72568,#72569,#72570,#72571,#72572));
#16241=EDGE_LOOP('',(#72573,#72574,#72575,#72576));
#16242=EDGE_LOOP('',(#72577,#72578,#72579,#72580));
#16243=EDGE_LOOP('',(#72581,#72582,#72583,#72584,#72585));
#16244=EDGE_LOOP('',(#72586,#72587,#72588,#72589));
#16245=EDGE_LOOP('',(#72590,#72591,#72592,#72593));
#16246=EDGE_LOOP('',(#72594,#72595,#72596,#72597));
#16247=EDGE_LOOP('',(#72598,#72599,#72600,#72601));
#16248=EDGE_LOOP('',(#72602,#72603,#72604,#72605,#72606));
#16249=EDGE_LOOP('',(#72607,#72608,#72609,#72610));
#16250=EDGE_LOOP('',(#72611,#72612,#72613,#72614));
#16251=EDGE_LOOP('',(#72615,#72616,#72617,#72618));
#16252=EDGE_LOOP('',(#72619,#72620,#72621,#72622));
#16253=EDGE_LOOP('',(#72623,#72624,#72625,#72626));
#16254=EDGE_LOOP('',(#72627,#72628,#72629,#72630));
#16255=EDGE_LOOP('',(#72631,#72632,#72633,#72634));
#16256=EDGE_LOOP('',(#72635,#72636,#72637,#72638));
#16257=EDGE_LOOP('',(#72639,#72640,#72641,#72642));
#16258=EDGE_LOOP('',(#72643,#72644,#72645,#72646));
#16259=EDGE_LOOP('',(#72647,#72648,#72649,#72650,#72651));
#16260=EDGE_LOOP('',(#72652,#72653,#72654,#72655));
#16261=EDGE_LOOP('',(#72656,#72657,#72658,#72659));
#16262=EDGE_LOOP('',(#72660,#72661,#72662,#72663));
#16263=EDGE_LOOP('',(#72664,#72665,#72666,#72667));
#16264=EDGE_LOOP('',(#72668,#72669,#72670,#72671));
#16265=EDGE_LOOP('',(#72672,#72673,#72674,#72675));
#16266=EDGE_LOOP('',(#72676,#72677,#72678,#72679));
#16267=EDGE_LOOP('',(#72680,#72681,#72682,#72683));
#16268=EDGE_LOOP('',(#72684,#72685,#72686,#72687,#72688));
#16269=EDGE_LOOP('',(#72689,#72690,#72691,#72692));
#16270=EDGE_LOOP('',(#72693,#72694,#72695,#72696));
#16271=EDGE_LOOP('',(#72697,#72698,#72699,#72700,#72701));
#16272=EDGE_LOOP('',(#72702,#72703,#72704,#72705));
#16273=EDGE_LOOP('',(#72706,#72707,#72708,#72709));
#16274=EDGE_LOOP('',(#72710,#72711,#72712,#72713));
#16275=EDGE_LOOP('',(#72714,#72715,#72716,#72717));
#16276=EDGE_LOOP('',(#72718,#72719,#72720,#72721,#72722));
#16277=EDGE_LOOP('',(#72723,#72724,#72725,#72726));
#16278=EDGE_LOOP('',(#72727,#72728,#72729,#72730));
#16279=EDGE_LOOP('',(#72731,#72732,#72733,#72734));
#16280=EDGE_LOOP('',(#72735,#72736,#72737,#72738));
#16281=EDGE_LOOP('',(#72739,#72740,#72741,#72742));
#16282=EDGE_LOOP('',(#72743,#72744,#72745,#72746));
#16283=EDGE_LOOP('',(#72747,#72748,#72749,#72750));
#16284=EDGE_LOOP('',(#72751,#72752,#72753,#72754));
#16285=EDGE_LOOP('',(#72755,#72756,#72757,#72758));
#16286=EDGE_LOOP('',(#72759,#72760,#72761,#72762));
#16287=EDGE_LOOP('',(#72763,#72764,#72765,#72766,#72767));
#16288=EDGE_LOOP('',(#72768,#72769,#72770,#72771));
#16289=EDGE_LOOP('',(#72772,#72773,#72774,#72775));
#16290=EDGE_LOOP('',(#72776,#72777,#72778,#72779));
#16291=EDGE_LOOP('',(#72780,#72781,#72782,#72783));
#16292=EDGE_LOOP('',(#72784,#72785,#72786,#72787));
#16293=EDGE_LOOP('',(#72788,#72789,#72790,#72791));
#16294=EDGE_LOOP('',(#72792,#72793,#72794,#72795));
#16295=EDGE_LOOP('',(#72796,#72797,#72798,#72799));
#16296=EDGE_LOOP('',(#72800,#72801,#72802,#72803,#72804));
#16297=EDGE_LOOP('',(#72805,#72806,#72807,#72808));
#16298=EDGE_LOOP('',(#72809,#72810,#72811,#72812));
#16299=EDGE_LOOP('',(#72813,#72814,#72815,#72816,#72817));
#16300=EDGE_LOOP('',(#72818,#72819,#72820,#72821));
#16301=EDGE_LOOP('',(#72822,#72823,#72824,#72825));
#16302=EDGE_LOOP('',(#72826,#72827,#72828,#72829));
#16303=EDGE_LOOP('',(#72830,#72831,#72832,#72833));
#16304=EDGE_LOOP('',(#72834,#72835,#72836,#72837,#72838));
#16305=EDGE_LOOP('',(#72839,#72840,#72841,#72842));
#16306=EDGE_LOOP('',(#72843,#72844,#72845,#72846));
#16307=EDGE_LOOP('',(#72847,#72848,#72849,#72850));
#16308=EDGE_LOOP('',(#72851,#72852,#72853,#72854));
#16309=EDGE_LOOP('',(#72855,#72856,#72857,#72858));
#16310=EDGE_LOOP('',(#72859,#72860,#72861,#72862));
#16311=EDGE_LOOP('',(#72863,#72864,#72865,#72866));
#16312=EDGE_LOOP('',(#72867,#72868,#72869,#72870));
#16313=EDGE_LOOP('',(#72871,#72872,#72873,#72874));
#16314=EDGE_LOOP('',(#72875,#72876,#72877,#72878));
#16315=EDGE_LOOP('',(#72879,#72880,#72881,#72882,#72883));
#16316=EDGE_LOOP('',(#72884,#72885,#72886,#72887));
#16317=EDGE_LOOP('',(#72888,#72889,#72890,#72891));
#16318=EDGE_LOOP('',(#72892,#72893,#72894,#72895));
#16319=EDGE_LOOP('',(#72896,#72897,#72898,#72899));
#16320=EDGE_LOOP('',(#72900,#72901,#72902,#72903));
#16321=EDGE_LOOP('',(#72904,#72905,#72906,#72907));
#16322=EDGE_LOOP('',(#72908,#72909,#72910,#72911));
#16323=EDGE_LOOP('',(#72912,#72913,#72914,#72915));
#16324=EDGE_LOOP('',(#72916,#72917,#72918,#72919,#72920));
#16325=EDGE_LOOP('',(#72921,#72922,#72923,#72924));
#16326=EDGE_LOOP('',(#72925,#72926,#72927,#72928));
#16327=EDGE_LOOP('',(#72929,#72930,#72931,#72932,#72933));
#16328=EDGE_LOOP('',(#72934,#72935,#72936,#72937));
#16329=EDGE_LOOP('',(#72938,#72939,#72940,#72941));
#16330=EDGE_LOOP('',(#72942,#72943,#72944,#72945));
#16331=EDGE_LOOP('',(#72946,#72947,#72948,#72949));
#16332=EDGE_LOOP('',(#72950,#72951,#72952,#72953,#72954));
#16333=EDGE_LOOP('',(#72955,#72956,#72957,#72958));
#16334=EDGE_LOOP('',(#72959,#72960,#72961,#72962));
#16335=EDGE_LOOP('',(#72963,#72964,#72965,#72966));
#16336=EDGE_LOOP('',(#72967,#72968,#72969,#72970));
#16337=EDGE_LOOP('',(#72971,#72972,#72973,#72974));
#16338=EDGE_LOOP('',(#72975,#72976,#72977,#72978));
#16339=EDGE_LOOP('',(#72979,#72980,#72981,#72982));
#16340=EDGE_LOOP('',(#72983,#72984,#72985,#72986));
#16341=EDGE_LOOP('',(#72987,#72988,#72989,#72990));
#16342=EDGE_LOOP('',(#72991,#72992,#72993,#72994));
#16343=EDGE_LOOP('',(#72995,#72996,#72997,#72998,#72999));
#16344=EDGE_LOOP('',(#73000,#73001,#73002,#73003));
#16345=EDGE_LOOP('',(#73004,#73005,#73006,#73007));
#16346=EDGE_LOOP('',(#73008,#73009,#73010,#73011));
#16347=EDGE_LOOP('',(#73012,#73013,#73014,#73015));
#16348=EDGE_LOOP('',(#73016,#73017,#73018,#73019));
#16349=EDGE_LOOP('',(#73020,#73021,#73022,#73023));
#16350=EDGE_LOOP('',(#73024,#73025,#73026,#73027));
#16351=EDGE_LOOP('',(#73028,#73029,#73030,#73031));
#16352=EDGE_LOOP('',(#73032,#73033,#73034,#73035,#73036));
#16353=EDGE_LOOP('',(#73037,#73038,#73039,#73040));
#16354=EDGE_LOOP('',(#73041,#73042,#73043,#73044));
#16355=EDGE_LOOP('',(#73045,#73046,#73047,#73048,#73049));
#16356=EDGE_LOOP('',(#73050,#73051,#73052,#73053));
#16357=EDGE_LOOP('',(#73054,#73055,#73056,#73057));
#16358=EDGE_LOOP('',(#73058,#73059,#73060,#73061));
#16359=EDGE_LOOP('',(#73062,#73063,#73064,#73065));
#16360=EDGE_LOOP('',(#73066,#73067,#73068,#73069,#73070));
#16361=EDGE_LOOP('',(#73071,#73072,#73073,#73074));
#16362=EDGE_LOOP('',(#73075,#73076,#73077,#73078));
#16363=EDGE_LOOP('',(#73079,#73080,#73081,#73082));
#16364=EDGE_LOOP('',(#73083,#73084,#73085,#73086));
#16365=EDGE_LOOP('',(#73087,#73088,#73089,#73090));
#16366=EDGE_LOOP('',(#73091,#73092,#73093,#73094));
#16367=EDGE_LOOP('',(#73095,#73096,#73097,#73098));
#16368=EDGE_LOOP('',(#73099,#73100,#73101,#73102));
#16369=EDGE_LOOP('',(#73103,#73104,#73105,#73106));
#16370=EDGE_LOOP('',(#73107,#73108,#73109,#73110));
#16371=EDGE_LOOP('',(#73111,#73112,#73113,#73114,#73115));
#16372=EDGE_LOOP('',(#73116,#73117,#73118,#73119));
#16373=EDGE_LOOP('',(#73120,#73121,#73122,#73123));
#16374=EDGE_LOOP('',(#73124,#73125,#73126,#73127));
#16375=EDGE_LOOP('',(#73128,#73129,#73130,#73131));
#16376=EDGE_LOOP('',(#73132,#73133,#73134,#73135));
#16377=EDGE_LOOP('',(#73136,#73137,#73138,#73139));
#16378=EDGE_LOOP('',(#73140,#73141,#73142,#73143));
#16379=EDGE_LOOP('',(#73144,#73145,#73146,#73147));
#16380=EDGE_LOOP('',(#73148,#73149,#73150,#73151,#73152));
#16381=EDGE_LOOP('',(#73153,#73154,#73155,#73156));
#16382=EDGE_LOOP('',(#73157,#73158,#73159,#73160));
#16383=EDGE_LOOP('',(#73161,#73162,#73163,#73164,#73165));
#16384=EDGE_LOOP('',(#73166,#73167,#73168,#73169));
#16385=EDGE_LOOP('',(#73170,#73171,#73172,#73173));
#16386=EDGE_LOOP('',(#73174,#73175,#73176,#73177));
#16387=EDGE_LOOP('',(#73178,#73179,#73180,#73181));
#16388=EDGE_LOOP('',(#73182,#73183,#73184,#73185,#73186));
#16389=EDGE_LOOP('',(#73187,#73188,#73189,#73190));
#16390=EDGE_LOOP('',(#73191,#73192,#73193,#73194));
#16391=EDGE_LOOP('',(#73195,#73196,#73197,#73198));
#16392=EDGE_LOOP('',(#73199,#73200,#73201,#73202));
#16393=EDGE_LOOP('',(#73203,#73204,#73205,#73206));
#16394=EDGE_LOOP('',(#73207,#73208,#73209,#73210));
#16395=EDGE_LOOP('',(#73211,#73212,#73213,#73214));
#16396=EDGE_LOOP('',(#73215,#73216,#73217,#73218));
#16397=EDGE_LOOP('',(#73219,#73220,#73221,#73222));
#16398=EDGE_LOOP('',(#73223,#73224,#73225,#73226));
#16399=EDGE_LOOP('',(#73227,#73228,#73229,#73230,#73231));
#16400=EDGE_LOOP('',(#73232,#73233,#73234,#73235));
#16401=EDGE_LOOP('',(#73236,#73237,#73238,#73239));
#16402=EDGE_LOOP('',(#73240,#73241,#73242,#73243));
#16403=EDGE_LOOP('',(#73244,#73245,#73246,#73247));
#16404=EDGE_LOOP('',(#73248,#73249,#73250,#73251));
#16405=EDGE_LOOP('',(#73252,#73253,#73254,#73255));
#16406=EDGE_LOOP('',(#73256,#73257,#73258,#73259));
#16407=EDGE_LOOP('',(#73260,#73261,#73262,#73263));
#16408=EDGE_LOOP('',(#73264,#73265,#73266,#73267,#73268));
#16409=EDGE_LOOP('',(#73269,#73270,#73271,#73272));
#16410=EDGE_LOOP('',(#73273,#73274,#73275,#73276));
#16411=EDGE_LOOP('',(#73277,#73278,#73279,#73280,#73281));
#16412=EDGE_LOOP('',(#73282,#73283,#73284,#73285));
#16413=EDGE_LOOP('',(#73286,#73287,#73288,#73289));
#16414=EDGE_LOOP('',(#73290,#73291,#73292,#73293));
#16415=EDGE_LOOP('',(#73294,#73295,#73296,#73297));
#16416=EDGE_LOOP('',(#73298,#73299,#73300,#73301,#73302));
#16417=EDGE_LOOP('',(#73303,#73304,#73305,#73306));
#16418=EDGE_LOOP('',(#73307,#73308,#73309,#73310));
#16419=EDGE_LOOP('',(#73311,#73312,#73313,#73314));
#16420=EDGE_LOOP('',(#73315,#73316,#73317,#73318));
#16421=EDGE_LOOP('',(#73319,#73320,#73321,#73322));
#16422=EDGE_LOOP('',(#73323,#73324,#73325,#73326));
#16423=EDGE_LOOP('',(#73327,#73328,#73329,#73330));
#16424=EDGE_LOOP('',(#73331,#73332,#73333,#73334));
#16425=EDGE_LOOP('',(#73335,#73336,#73337,#73338));
#16426=EDGE_LOOP('',(#73339,#73340,#73341,#73342));
#16427=EDGE_LOOP('',(#73343,#73344,#73345,#73346,#73347));
#16428=EDGE_LOOP('',(#73348,#73349,#73350,#73351));
#16429=EDGE_LOOP('',(#73352,#73353,#73354,#73355));
#16430=EDGE_LOOP('',(#73356,#73357,#73358,#73359));
#16431=EDGE_LOOP('',(#73360,#73361,#73362,#73363));
#16432=EDGE_LOOP('',(#73364,#73365,#73366,#73367));
#16433=EDGE_LOOP('',(#73368,#73369,#73370,#73371));
#16434=EDGE_LOOP('',(#73372,#73373,#73374,#73375));
#16435=EDGE_LOOP('',(#73376,#73377,#73378,#73379));
#16436=EDGE_LOOP('',(#73380,#73381,#73382,#73383,#73384));
#16437=EDGE_LOOP('',(#73385,#73386,#73387,#73388));
#16438=EDGE_LOOP('',(#73389,#73390,#73391,#73392));
#16439=EDGE_LOOP('',(#73393,#73394,#73395,#73396,#73397));
#16440=EDGE_LOOP('',(#73398,#73399,#73400,#73401));
#16441=EDGE_LOOP('',(#73402,#73403,#73404,#73405));
#16442=EDGE_LOOP('',(#73406,#73407,#73408,#73409));
#16443=EDGE_LOOP('',(#73410,#73411,#73412,#73413));
#16444=EDGE_LOOP('',(#73414,#73415,#73416,#73417,#73418));
#16445=EDGE_LOOP('',(#73419,#73420,#73421,#73422));
#16446=EDGE_LOOP('',(#73423,#73424,#73425,#73426));
#16447=EDGE_LOOP('',(#73427,#73428,#73429,#73430));
#16448=EDGE_LOOP('',(#73431,#73432,#73433,#73434));
#16449=EDGE_LOOP('',(#73435,#73436,#73437,#73438));
#16450=EDGE_LOOP('',(#73439,#73440,#73441,#73442));
#16451=EDGE_LOOP('',(#73443,#73444,#73445,#73446));
#16452=EDGE_LOOP('',(#73447,#73448,#73449,#73450));
#16453=EDGE_LOOP('',(#73451,#73452,#73453,#73454));
#16454=EDGE_LOOP('',(#73455,#73456,#73457,#73458));
#16455=EDGE_LOOP('',(#73459,#73460,#73461,#73462,#73463));
#16456=EDGE_LOOP('',(#73464,#73465,#73466,#73467));
#16457=EDGE_LOOP('',(#73468,#73469,#73470,#73471));
#16458=EDGE_LOOP('',(#73472,#73473,#73474,#73475));
#16459=EDGE_LOOP('',(#73476,#73477,#73478,#73479));
#16460=EDGE_LOOP('',(#73480,#73481,#73482,#73483));
#16461=EDGE_LOOP('',(#73484,#73485,#73486,#73487));
#16462=EDGE_LOOP('',(#73488,#73489,#73490,#73491));
#16463=EDGE_LOOP('',(#73492,#73493,#73494,#73495));
#16464=EDGE_LOOP('',(#73496,#73497,#73498,#73499,#73500));
#16465=EDGE_LOOP('',(#73501,#73502,#73503,#73504));
#16466=EDGE_LOOP('',(#73505,#73506,#73507,#73508));
#16467=EDGE_LOOP('',(#73509,#73510,#73511,#73512));
#16468=EDGE_LOOP('',(#73513,#73514,#73515,#73516,#73517));
#16469=EDGE_LOOP('',(#73518,#73519,#73520,#73521,#73522));
#16470=EDGE_LOOP('',(#73523,#73524,#73525,#73526));
#16471=EDGE_LOOP('',(#73527,#73528,#73529,#73530,#73531));
#16472=EDGE_LOOP('',(#73532,#73533,#73534,#73535));
#16473=EDGE_LOOP('',(#73536,#73537,#73538,#73539));
#16474=EDGE_LOOP('',(#73540,#73541,#73542,#73543));
#16475=EDGE_LOOP('',(#73544,#73545,#73546,#73547,#73548,#73549,#73550,#73551,
#73552,#73553,#73554,#73555,#73556,#73557,#73558,#73559,#73560,#73561,#73562,
#73563,#73564,#73565,#73566,#73567,#73568,#73569,#73570,#73571,#73572,#73573,
#73574,#73575,#73576,#73577,#73578,#73579,#73580,#73581,#73582,#73583,#73584,
#73585,#73586,#73587,#73588,#73589,#73590,#73591,#73592,#73593,#73594,#73595,
#73596,#73597,#73598,#73599,#73600,#73601,#73602,#73603,#73604,#73605,#73606,
#73607,#73608,#73609,#73610,#73611,#73612,#73613,#73614,#73615,#73616,#73617,
#73618,#73619,#73620,#73621,#73622,#73623,#73624,#73625,#73626,#73627,#73628,
#73629,#73630,#73631,#73632,#73633,#73634,#73635,#73636,#73637,#73638,#73639,
#73640,#73641,#73642,#73643,#73644,#73645,#73646,#73647,#73648,#73649,#73650,
#73651,#73652,#73653,#73654,#73655,#73656,#73657,#73658,#73659,#73660,#73661,
#73662,#73663,#73664,#73665,#73666,#73667,#73668,#73669,#73670,#73671,#73672,
#73673,#73674,#73675,#73676,#73677,#73678,#73679,#73680,#73681,#73682,#73683,
#73684,#73685,#73686,#73687,#73688,#73689,#73690,#73691,#73692,#73693,#73694,
#73695,#73696,#73697,#73698,#73699,#73700,#73701,#73702,#73703,#73704,#73705,
#73706,#73707,#73708,#73709,#73710,#73711,#73712,#73713,#73714,#73715,#73716,
#73717,#73718,#73719,#73720,#73721,#73722,#73723,#73724,#73725,#73726,#73727,
#73728,#73729,#73730,#73731,#73732,#73733,#73734,#73735,#73736,#73737,#73738,
#73739,#73740,#73741,#73742,#73743,#73744,#73745,#73746,#73747,#73748,#73749,
#73750,#73751,#73752,#73753,#73754,#73755,#73756,#73757,#73758,#73759,#73760,
#73761,#73762,#73763,#73764,#73765,#73766,#73767,#73768,#73769,#73770,#73771,
#73772,#73773,#73774,#73775,#73776,#73777,#73778,#73779,#73780,#73781,#73782,
#73783,#73784,#73785,#73786,#73787,#73788,#73789,#73790,#73791,#73792,#73793,
#73794,#73795,#73796,#73797,#73798,#73799,#73800,#73801,#73802,#73803,#73804,
#73805,#73806,#73807,#73808,#73809,#73810,#73811,#73812,#73813,#73814,#73815,
#73816,#73817,#73818,#73819,#73820,#73821,#73822,#73823,#73824,#73825,#73826,
#73827,#73828,#73829,#73830,#73831,#73832,#73833,#73834,#73835,#73836,#73837,
#73838,#73839,#73840,#73841,#73842,#73843,#73844,#73845,#73846,#73847,#73848,
#73849,#73850,#73851,#73852,#73853,#73854,#73855,#73856,#73857,#73858,#73859,
#73860,#73861,#73862,#73863,#73864,#73865,#73866,#73867,#73868,#73869,#73870,
#73871,#73872,#73873,#73874,#73875,#73876,#73877,#73878,#73879,#73880,#73881,
#73882,#73883,#73884,#73885,#73886,#73887,#73888,#73889,#73890,#73891,#73892,
#73893,#73894,#73895,#73896,#73897,#73898,#73899,#73900,#73901,#73902,#73903,
#73904,#73905,#73906,#73907,#73908));
#16476=EDGE_LOOP('',(#73909,#73910,#73911,#73912,#73913,#73914,#73915,#73916,
#73917,#73918,#73919,#73920,#73921,#73922,#73923,#73924,#73925,#73926,#73927,
#73928,#73929,#73930,#73931,#73932,#73933,#73934,#73935,#73936,#73937,#73938,
#73939,#73940,#73941,#73942,#73943,#73944,#73945,#73946,#73947,#73948,#73949,
#73950,#73951,#73952,#73953,#73954,#73955,#73956,#73957,#73958,#73959,#73960,
#73961,#73962,#73963,#73964,#73965,#73966,#73967,#73968,#73969,#73970,#73971,
#73972,#73973,#73974,#73975,#73976,#73977,#73978,#73979,#73980,#73981,#73982,
#73983,#73984,#73985,#73986,#73987,#73988,#73989,#73990,#73991,#73992,#73993,
#73994,#73995,#73996,#73997,#73998,#73999,#74000,#74001,#74002,#74003,#74004,
#74005,#74006,#74007,#74008,#74009,#74010,#74011,#74012,#74013,#74014,#74015,
#74016,#74017,#74018,#74019,#74020,#74021,#74022,#74023,#74024,#74025,#74026,
#74027,#74028,#74029,#74030,#74031,#74032,#74033,#74034,#74035,#74036,#74037,
#74038,#74039,#74040,#74041,#74042,#74043,#74044,#74045,#74046,#74047,#74048,
#74049,#74050,#74051,#74052,#74053,#74054,#74055,#74056,#74057,#74058,#74059,
#74060,#74061,#74062,#74063,#74064,#74065,#74066,#74067,#74068,#74069,#74070,
#74071,#74072,#74073,#74074,#74075,#74076,#74077,#74078,#74079,#74080,#74081,
#74082,#74083,#74084,#74085,#74086,#74087,#74088,#74089,#74090,#74091,#74092,
#74093,#74094,#74095,#74096,#74097,#74098,#74099,#74100,#74101,#74102,#74103,
#74104,#74105,#74106,#74107,#74108,#74109,#74110,#74111,#74112,#74113,#74114,
#74115,#74116,#74117,#74118,#74119,#74120,#74121,#74122,#74123,#74124,#74125,
#74126,#74127,#74128,#74129,#74130,#74131,#74132,#74133,#74134,#74135,#74136,
#74137,#74138,#74139,#74140,#74141,#74142,#74143,#74144,#74145,#74146,#74147,
#74148,#74149,#74150,#74151,#74152,#74153,#74154,#74155,#74156,#74157,#74158,
#74159,#74160,#74161,#74162,#74163,#74164,#74165,#74166,#74167,#74168,#74169,
#74170,#74171,#74172,#74173,#74174,#74175,#74176,#74177,#74178,#74179,#74180,
#74181,#74182,#74183,#74184,#74185,#74186,#74187,#74188,#74189,#74190,#74191,
#74192,#74193,#74194,#74195,#74196,#74197,#74198,#74199,#74200,#74201,#74202,
#74203,#74204,#74205,#74206,#74207,#74208,#74209,#74210,#74211,#74212,#74213,
#74214,#74215,#74216,#74217,#74218,#74219,#74220,#74221,#74222,#74223,#74224,
#74225,#74226,#74227,#74228,#74229,#74230,#74231,#74232,#74233,#74234,#74235,
#74236,#74237,#74238,#74239,#74240,#74241,#74242,#74243,#74244,#74245,#74246,
#74247,#74248,#74249,#74250,#74251,#74252,#74253,#74254,#74255,#74256,#74257,
#74258,#74259,#74260,#74261,#74262,#74263,#74264,#74265,#74266,#74267,#74268,
#74269,#74270,#74271,#74272));
#16477=EDGE_LOOP('',(#74273,#74274,#74275,#74276,#74277,#74278));
#16478=EDGE_LOOP('',(#74279,#74280,#74281,#74282,#74283));
#16479=EDGE_LOOP('',(#74284,#74285,#74286,#74287,#74288,#74289));
#16480=EDGE_LOOP('',(#74290,#74291,#74292,#74293));
#16481=EDGE_LOOP('',(#74294,#74295,#74296,#74297));
#16482=EDGE_LOOP('',(#74298,#74299,#74300,#74301,#74302,#74303));
#16483=EDGE_LOOP('',(#74304,#74305,#74306,#74307));
#16484=EDGE_LOOP('',(#74308,#74309,#74310,#74311));
#16485=EDGE_LOOP('',(#74312,#74313,#74314,#74315));
#16486=EDGE_LOOP('',(#74316,#74317,#74318,#74319));
#16487=EDGE_LOOP('',(#74320,#74321,#74322,#74323));
#16488=EDGE_LOOP('',(#74324,#74325,#74326,#74327,#74328,#74329));
#16489=EDGE_LOOP('',(#74330,#74331,#74332,#74333));
#16490=EDGE_LOOP('',(#74334,#74335,#74336,#74337));
#16491=EDGE_LOOP('',(#74338,#74339,#74340,#74341,#74342,#74343));
#16492=EDGE_LOOP('',(#74344,#74345,#74346,#74347));
#16493=EDGE_LOOP('',(#74348,#74349,#74350,#74351));
#16494=EDGE_LOOP('',(#74352,#74353,#74354,#74355));
#16495=EDGE_LOOP('',(#74356,#74357,#74358,#74359));
#16496=EDGE_LOOP('',(#74360,#74361,#74362,#74363));
#16497=EDGE_LOOP('',(#74364,#74365,#74366,#74367,#74368,#74369));
#16498=EDGE_LOOP('',(#74370,#74371,#74372,#74373));
#16499=EDGE_LOOP('',(#74374,#74375,#74376,#74377));
#16500=EDGE_LOOP('',(#74378,#74379,#74380,#74381,#74382,#74383));
#16501=EDGE_LOOP('',(#74384,#74385,#74386,#74387));
#16502=EDGE_LOOP('',(#74388,#74389,#74390,#74391));
#16503=EDGE_LOOP('',(#74392,#74393,#74394,#74395));
#16504=EDGE_LOOP('',(#74396,#74397,#74398,#74399));
#16505=EDGE_LOOP('',(#74400,#74401,#74402,#74403));
#16506=EDGE_LOOP('',(#74404,#74405,#74406,#74407,#74408,#74409));
#16507=EDGE_LOOP('',(#74410,#74411,#74412,#74413));
#16508=EDGE_LOOP('',(#74414,#74415,#74416,#74417));
#16509=EDGE_LOOP('',(#74418,#74419,#74420,#74421,#74422,#74423));
#16510=EDGE_LOOP('',(#74424,#74425,#74426,#74427));
#16511=EDGE_LOOP('',(#74428,#74429,#74430,#74431));
#16512=EDGE_LOOP('',(#74432,#74433,#74434,#74435));
#16513=EDGE_LOOP('',(#74436,#74437,#74438,#74439));
#16514=EDGE_LOOP('',(#74440,#74441,#74442,#74443));
#16515=EDGE_LOOP('',(#74444,#74445,#74446,#74447,#74448,#74449));
#16516=EDGE_LOOP('',(#74450,#74451,#74452,#74453));
#16517=EDGE_LOOP('',(#74454,#74455,#74456,#74457));
#16518=EDGE_LOOP('',(#74458,#74459,#74460,#74461,#74462,#74463));
#16519=EDGE_LOOP('',(#74464,#74465,#74466,#74467));
#16520=EDGE_LOOP('',(#74468,#74469,#74470,#74471));
#16521=EDGE_LOOP('',(#74472,#74473,#74474,#74475));
#16522=EDGE_LOOP('',(#74476,#74477,#74478,#74479));
#16523=EDGE_LOOP('',(#74480,#74481,#74482,#74483));
#16524=EDGE_LOOP('',(#74484,#74485,#74486,#74487,#74488,#74489));
#16525=EDGE_LOOP('',(#74490,#74491,#74492,#74493));
#16526=EDGE_LOOP('',(#74494,#74495,#74496,#74497));
#16527=EDGE_LOOP('',(#74498,#74499,#74500,#74501,#74502,#74503));
#16528=EDGE_LOOP('',(#74504,#74505,#74506,#74507));
#16529=EDGE_LOOP('',(#74508,#74509,#74510,#74511));
#16530=EDGE_LOOP('',(#74512,#74513,#74514,#74515));
#16531=EDGE_LOOP('',(#74516,#74517,#74518,#74519));
#16532=EDGE_LOOP('',(#74520,#74521,#74522,#74523));
#16533=EDGE_LOOP('',(#74524,#74525,#74526,#74527,#74528,#74529));
#16534=EDGE_LOOP('',(#74530,#74531,#74532,#74533));
#16535=EDGE_LOOP('',(#74534,#74535,#74536,#74537));
#16536=EDGE_LOOP('',(#74538,#74539,#74540,#74541,#74542,#74543));
#16537=EDGE_LOOP('',(#74544,#74545,#74546,#74547));
#16538=EDGE_LOOP('',(#74548,#74549,#74550,#74551));
#16539=EDGE_LOOP('',(#74552,#74553,#74554,#74555));
#16540=EDGE_LOOP('',(#74556,#74557,#74558,#74559));
#16541=EDGE_LOOP('',(#74560,#74561,#74562,#74563));
#16542=EDGE_LOOP('',(#74564,#74565,#74566,#74567,#74568,#74569));
#16543=EDGE_LOOP('',(#74570,#74571,#74572,#74573));
#16544=EDGE_LOOP('',(#74574,#74575,#74576,#74577));
#16545=EDGE_LOOP('',(#74578,#74579,#74580,#74581,#74582,#74583));
#16546=EDGE_LOOP('',(#74584,#74585,#74586,#74587));
#16547=EDGE_LOOP('',(#74588,#74589,#74590,#74591));
#16548=EDGE_LOOP('',(#74592,#74593,#74594,#74595));
#16549=EDGE_LOOP('',(#74596,#74597,#74598,#74599));
#16550=EDGE_LOOP('',(#74600,#74601,#74602,#74603));
#16551=EDGE_LOOP('',(#74604,#74605,#74606,#74607,#74608,#74609));
#16552=EDGE_LOOP('',(#74610,#74611,#74612,#74613));
#16553=EDGE_LOOP('',(#74614,#74615,#74616,#74617));
#16554=EDGE_LOOP('',(#74618,#74619,#74620,#74621,#74622,#74623));
#16555=EDGE_LOOP('',(#74624,#74625,#74626,#74627));
#16556=EDGE_LOOP('',(#74628,#74629,#74630,#74631));
#16557=EDGE_LOOP('',(#74632,#74633,#74634,#74635));
#16558=EDGE_LOOP('',(#74636,#74637,#74638,#74639));
#16559=EDGE_LOOP('',(#74640,#74641,#74642,#74643));
#16560=EDGE_LOOP('',(#74644,#74645,#74646,#74647,#74648,#74649));
#16561=EDGE_LOOP('',(#74650,#74651,#74652,#74653));
#16562=EDGE_LOOP('',(#74654,#74655,#74656,#74657));
#16563=EDGE_LOOP('',(#74658,#74659,#74660,#74661,#74662,#74663));
#16564=EDGE_LOOP('',(#74664,#74665,#74666,#74667));
#16565=EDGE_LOOP('',(#74668,#74669,#74670,#74671));
#16566=EDGE_LOOP('',(#74672,#74673,#74674,#74675));
#16567=EDGE_LOOP('',(#74676,#74677,#74678,#74679));
#16568=EDGE_LOOP('',(#74680,#74681,#74682,#74683));
#16569=EDGE_LOOP('',(#74684,#74685,#74686,#74687,#74688,#74689));
#16570=EDGE_LOOP('',(#74690,#74691,#74692,#74693));
#16571=EDGE_LOOP('',(#74694,#74695,#74696,#74697));
#16572=EDGE_LOOP('',(#74698,#74699,#74700,#74701,#74702,#74703));
#16573=EDGE_LOOP('',(#74704,#74705,#74706,#74707));
#16574=EDGE_LOOP('',(#74708,#74709,#74710,#74711));
#16575=EDGE_LOOP('',(#74712,#74713,#74714,#74715));
#16576=EDGE_LOOP('',(#74716,#74717,#74718,#74719));
#16577=EDGE_LOOP('',(#74720,#74721,#74722,#74723));
#16578=EDGE_LOOP('',(#74724,#74725,#74726,#74727,#74728,#74729));
#16579=EDGE_LOOP('',(#74730,#74731,#74732,#74733));
#16580=EDGE_LOOP('',(#74734,#74735,#74736,#74737));
#16581=EDGE_LOOP('',(#74738,#74739,#74740,#74741,#74742,#74743));
#16582=EDGE_LOOP('',(#74744,#74745,#74746,#74747));
#16583=EDGE_LOOP('',(#74748,#74749,#74750,#74751));
#16584=EDGE_LOOP('',(#74752,#74753,#74754,#74755));
#16585=EDGE_LOOP('',(#74756,#74757,#74758,#74759));
#16586=EDGE_LOOP('',(#74760,#74761,#74762,#74763));
#16587=EDGE_LOOP('',(#74764,#74765,#74766,#74767,#74768,#74769));
#16588=EDGE_LOOP('',(#74770,#74771,#74772,#74773));
#16589=EDGE_LOOP('',(#74774,#74775,#74776,#74777));
#16590=EDGE_LOOP('',(#74778,#74779,#74780,#74781,#74782,#74783));
#16591=EDGE_LOOP('',(#74784,#74785,#74786,#74787));
#16592=EDGE_LOOP('',(#74788,#74789,#74790,#74791));
#16593=EDGE_LOOP('',(#74792,#74793,#74794,#74795));
#16594=EDGE_LOOP('',(#74796,#74797,#74798,#74799));
#16595=EDGE_LOOP('',(#74800,#74801,#74802,#74803));
#16596=EDGE_LOOP('',(#74804,#74805,#74806,#74807,#74808,#74809));
#16597=EDGE_LOOP('',(#74810,#74811,#74812,#74813));
#16598=EDGE_LOOP('',(#74814,#74815,#74816,#74817));
#16599=EDGE_LOOP('',(#74818,#74819,#74820,#74821,#74822,#74823));
#16600=EDGE_LOOP('',(#74824,#74825,#74826,#74827));
#16601=EDGE_LOOP('',(#74828,#74829,#74830,#74831));
#16602=EDGE_LOOP('',(#74832,#74833,#74834,#74835));
#16603=EDGE_LOOP('',(#74836,#74837,#74838,#74839));
#16604=EDGE_LOOP('',(#74840,#74841,#74842,#74843));
#16605=EDGE_LOOP('',(#74844,#74845,#74846,#74847,#74848,#74849));
#16606=EDGE_LOOP('',(#74850,#74851,#74852,#74853));
#16607=EDGE_LOOP('',(#74854,#74855,#74856,#74857));
#16608=EDGE_LOOP('',(#74858,#74859,#74860,#74861,#74862,#74863));
#16609=EDGE_LOOP('',(#74864,#74865,#74866,#74867));
#16610=EDGE_LOOP('',(#74868,#74869,#74870,#74871));
#16611=EDGE_LOOP('',(#74872,#74873,#74874,#74875));
#16612=EDGE_LOOP('',(#74876,#74877,#74878,#74879));
#16613=EDGE_LOOP('',(#74880,#74881,#74882,#74883));
#16614=EDGE_LOOP('',(#74884,#74885,#74886,#74887,#74888,#74889));
#16615=EDGE_LOOP('',(#74890,#74891,#74892,#74893));
#16616=EDGE_LOOP('',(#74894,#74895,#74896,#74897));
#16617=EDGE_LOOP('',(#74898,#74899,#74900,#74901,#74902,#74903));
#16618=EDGE_LOOP('',(#74904,#74905,#74906,#74907));
#16619=EDGE_LOOP('',(#74908,#74909,#74910,#74911));
#16620=EDGE_LOOP('',(#74912,#74913,#74914,#74915));
#16621=EDGE_LOOP('',(#74916,#74917,#74918,#74919));
#16622=EDGE_LOOP('',(#74920,#74921,#74922,#74923));
#16623=EDGE_LOOP('',(#74924,#74925,#74926,#74927,#74928,#74929));
#16624=EDGE_LOOP('',(#74930,#74931,#74932,#74933));
#16625=EDGE_LOOP('',(#74934,#74935,#74936,#74937));
#16626=EDGE_LOOP('',(#74938,#74939,#74940,#74941,#74942,#74943));
#16627=EDGE_LOOP('',(#74944,#74945,#74946,#74947));
#16628=EDGE_LOOP('',(#74948,#74949,#74950,#74951));
#16629=EDGE_LOOP('',(#74952,#74953,#74954,#74955));
#16630=EDGE_LOOP('',(#74956,#74957,#74958,#74959));
#16631=EDGE_LOOP('',(#74960,#74961,#74962,#74963));
#16632=EDGE_LOOP('',(#74964,#74965,#74966,#74967,#74968,#74969));
#16633=EDGE_LOOP('',(#74970,#74971,#74972,#74973));
#16634=EDGE_LOOP('',(#74974,#74975,#74976,#74977));
#16635=EDGE_LOOP('',(#74978,#74979,#74980,#74981,#74982,#74983));
#16636=EDGE_LOOP('',(#74984,#74985,#74986,#74987));
#16637=EDGE_LOOP('',(#74988,#74989,#74990,#74991));
#16638=EDGE_LOOP('',(#74992,#74993,#74994,#74995));
#16639=EDGE_LOOP('',(#74996,#74997,#74998,#74999));
#16640=EDGE_LOOP('',(#75000,#75001,#75002,#75003));
#16641=EDGE_LOOP('',(#75004,#75005,#75006,#75007,#75008,#75009));
#16642=EDGE_LOOP('',(#75010,#75011,#75012,#75013));
#16643=EDGE_LOOP('',(#75014,#75015,#75016,#75017));
#16644=EDGE_LOOP('',(#75018,#75019,#75020,#75021,#75022,#75023));
#16645=EDGE_LOOP('',(#75024,#75025,#75026,#75027));
#16646=EDGE_LOOP('',(#75028,#75029,#75030,#75031));
#16647=EDGE_LOOP('',(#75032,#75033,#75034,#75035));
#16648=EDGE_LOOP('',(#75036,#75037,#75038,#75039));
#16649=EDGE_LOOP('',(#75040,#75041,#75042,#75043));
#16650=EDGE_LOOP('',(#75044,#75045,#75046,#75047,#75048,#75049));
#16651=EDGE_LOOP('',(#75050,#75051,#75052,#75053));
#16652=EDGE_LOOP('',(#75054,#75055,#75056,#75057));
#16653=EDGE_LOOP('',(#75058,#75059,#75060,#75061,#75062,#75063));
#16654=EDGE_LOOP('',(#75064,#75065,#75066,#75067));
#16655=EDGE_LOOP('',(#75068,#75069,#75070,#75071));
#16656=EDGE_LOOP('',(#75072,#75073,#75074,#75075));
#16657=EDGE_LOOP('',(#75076,#75077,#75078,#75079));
#16658=EDGE_LOOP('',(#75080,#75081,#75082,#75083));
#16659=EDGE_LOOP('',(#75084,#75085,#75086,#75087,#75088,#75089));
#16660=EDGE_LOOP('',(#75090,#75091,#75092,#75093));
#16661=EDGE_LOOP('',(#75094,#75095,#75096,#75097));
#16662=EDGE_LOOP('',(#75098,#75099,#75100,#75101,#75102,#75103));
#16663=EDGE_LOOP('',(#75104,#75105,#75106,#75107));
#16664=EDGE_LOOP('',(#75108,#75109,#75110,#75111));
#16665=EDGE_LOOP('',(#75112,#75113,#75114,#75115));
#16666=EDGE_LOOP('',(#75116,#75117,#75118,#75119));
#16667=EDGE_LOOP('',(#75120,#75121,#75122,#75123));
#16668=EDGE_LOOP('',(#75124,#75125,#75126,#75127,#75128,#75129));
#16669=EDGE_LOOP('',(#75130,#75131,#75132,#75133));
#16670=EDGE_LOOP('',(#75134,#75135,#75136,#75137));
#16671=EDGE_LOOP('',(#75138,#75139,#75140,#75141,#75142,#75143));
#16672=EDGE_LOOP('',(#75144,#75145,#75146,#75147));
#16673=EDGE_LOOP('',(#75148,#75149,#75150,#75151));
#16674=EDGE_LOOP('',(#75152,#75153,#75154,#75155));
#16675=EDGE_LOOP('',(#75156,#75157,#75158,#75159));
#16676=EDGE_LOOP('',(#75160,#75161,#75162,#75163));
#16677=EDGE_LOOP('',(#75164,#75165,#75166,#75167,#75168,#75169));
#16678=EDGE_LOOP('',(#75170,#75171,#75172,#75173));
#16679=EDGE_LOOP('',(#75174,#75175,#75176,#75177));
#16680=EDGE_LOOP('',(#75178,#75179,#75180,#75181,#75182,#75183));
#16681=EDGE_LOOP('',(#75184,#75185,#75186,#75187));
#16682=EDGE_LOOP('',(#75188,#75189,#75190,#75191));
#16683=EDGE_LOOP('',(#75192,#75193,#75194,#75195));
#16684=EDGE_LOOP('',(#75196,#75197,#75198,#75199));
#16685=EDGE_LOOP('',(#75200,#75201,#75202,#75203));
#16686=EDGE_LOOP('',(#75204,#75205,#75206,#75207,#75208,#75209));
#16687=EDGE_LOOP('',(#75210,#75211,#75212,#75213));
#16688=EDGE_LOOP('',(#75214,#75215,#75216,#75217));
#16689=EDGE_LOOP('',(#75218,#75219,#75220,#75221,#75222,#75223));
#16690=EDGE_LOOP('',(#75224,#75225,#75226,#75227));
#16691=EDGE_LOOP('',(#75228,#75229,#75230,#75231));
#16692=EDGE_LOOP('',(#75232,#75233,#75234,#75235));
#16693=EDGE_LOOP('',(#75236,#75237,#75238,#75239));
#16694=EDGE_LOOP('',(#75240,#75241,#75242,#75243));
#16695=EDGE_LOOP('',(#75244,#75245,#75246,#75247,#75248,#75249));
#16696=EDGE_LOOP('',(#75250,#75251,#75252,#75253));
#16697=EDGE_LOOP('',(#75254,#75255,#75256,#75257));
#16698=EDGE_LOOP('',(#75258,#75259,#75260,#75261,#75262,#75263));
#16699=EDGE_LOOP('',(#75264,#75265,#75266,#75267));
#16700=EDGE_LOOP('',(#75268,#75269,#75270,#75271));
#16701=EDGE_LOOP('',(#75272,#75273,#75274,#75275));
#16702=EDGE_LOOP('',(#75276,#75277,#75278,#75279));
#16703=EDGE_LOOP('',(#75280,#75281,#75282,#75283));
#16704=EDGE_LOOP('',(#75284,#75285,#75286,#75287,#75288,#75289));
#16705=EDGE_LOOP('',(#75290,#75291,#75292,#75293));
#16706=EDGE_LOOP('',(#75294,#75295,#75296,#75297));
#16707=EDGE_LOOP('',(#75298,#75299,#75300,#75301,#75302,#75303));
#16708=EDGE_LOOP('',(#75304,#75305,#75306,#75307));
#16709=EDGE_LOOP('',(#75308,#75309,#75310,#75311));
#16710=EDGE_LOOP('',(#75312,#75313,#75314,#75315));
#16711=EDGE_LOOP('',(#75316,#75317,#75318,#75319));
#16712=EDGE_LOOP('',(#75320,#75321,#75322,#75323));
#16713=EDGE_LOOP('',(#75324,#75325,#75326,#75327,#75328,#75329));
#16714=EDGE_LOOP('',(#75330,#75331,#75332,#75333));
#16715=EDGE_LOOP('',(#75334,#75335,#75336,#75337));
#16716=EDGE_LOOP('',(#75338,#75339,#75340,#75341,#75342,#75343));
#16717=EDGE_LOOP('',(#75344,#75345,#75346,#75347));
#16718=EDGE_LOOP('',(#75348,#75349,#75350,#75351));
#16719=EDGE_LOOP('',(#75352,#75353,#75354,#75355));
#16720=EDGE_LOOP('',(#75356,#75357,#75358,#75359));
#16721=EDGE_LOOP('',(#75360,#75361,#75362,#75363));
#16722=EDGE_LOOP('',(#75364,#75365,#75366,#75367,#75368,#75369));
#16723=EDGE_LOOP('',(#75370,#75371,#75372,#75373));
#16724=EDGE_LOOP('',(#75374,#75375,#75376,#75377));
#16725=EDGE_LOOP('',(#75378,#75379,#75380,#75381,#75382,#75383));
#16726=EDGE_LOOP('',(#75384,#75385,#75386,#75387));
#16727=EDGE_LOOP('',(#75388,#75389,#75390,#75391));
#16728=EDGE_LOOP('',(#75392,#75393,#75394,#75395));
#16729=EDGE_LOOP('',(#75396,#75397,#75398,#75399));
#16730=EDGE_LOOP('',(#75400,#75401,#75402,#75403));
#16731=EDGE_LOOP('',(#75404,#75405,#75406,#75407,#75408,#75409));
#16732=EDGE_LOOP('',(#75410,#75411,#75412,#75413));
#16733=EDGE_LOOP('',(#75414,#75415,#75416,#75417));
#16734=EDGE_LOOP('',(#75418,#75419,#75420,#75421,#75422,#75423));
#16735=EDGE_LOOP('',(#75424,#75425,#75426,#75427));
#16736=EDGE_LOOP('',(#75428,#75429,#75430,#75431));
#16737=EDGE_LOOP('',(#75432,#75433,#75434,#75435));
#16738=EDGE_LOOP('',(#75436,#75437,#75438,#75439));
#16739=EDGE_LOOP('',(#75440,#75441,#75442,#75443));
#16740=EDGE_LOOP('',(#75444,#75445,#75446,#75447,#75448,#75449));
#16741=EDGE_LOOP('',(#75450,#75451,#75452,#75453));
#16742=EDGE_LOOP('',(#75454,#75455,#75456,#75457));
#16743=EDGE_LOOP('',(#75458,#75459,#75460,#75461,#75462,#75463));
#16744=EDGE_LOOP('',(#75464,#75465,#75466,#75467));
#16745=EDGE_LOOP('',(#75468,#75469,#75470,#75471));
#16746=EDGE_LOOP('',(#75472,#75473,#75474,#75475));
#16747=EDGE_LOOP('',(#75476,#75477,#75478,#75479));
#16748=EDGE_LOOP('',(#75480,#75481,#75482,#75483));
#16749=EDGE_LOOP('',(#75484,#75485,#75486,#75487,#75488,#75489));
#16750=EDGE_LOOP('',(#75490,#75491,#75492,#75493));
#16751=EDGE_LOOP('',(#75494,#75495,#75496,#75497));
#16752=EDGE_LOOP('',(#75498,#75499,#75500,#75501,#75502,#75503));
#16753=EDGE_LOOP('',(#75504,#75505,#75506,#75507));
#16754=EDGE_LOOP('',(#75508,#75509,#75510,#75511));
#16755=EDGE_LOOP('',(#75512,#75513,#75514,#75515));
#16756=EDGE_LOOP('',(#75516,#75517,#75518,#75519));
#16757=EDGE_LOOP('',(#75520,#75521,#75522,#75523));
#16758=EDGE_LOOP('',(#75524,#75525,#75526,#75527,#75528,#75529));
#16759=EDGE_LOOP('',(#75530,#75531,#75532,#75533));
#16760=EDGE_LOOP('',(#75534,#75535,#75536,#75537));
#16761=EDGE_LOOP('',(#75538,#75539,#75540,#75541,#75542,#75543));
#16762=EDGE_LOOP('',(#75544,#75545,#75546,#75547));
#16763=EDGE_LOOP('',(#75548,#75549,#75550,#75551));
#16764=EDGE_LOOP('',(#75552,#75553,#75554,#75555));
#16765=EDGE_LOOP('',(#75556,#75557,#75558,#75559));
#16766=EDGE_LOOP('',(#75560,#75561,#75562,#75563));
#16767=EDGE_LOOP('',(#75564,#75565,#75566,#75567,#75568,#75569));
#16768=EDGE_LOOP('',(#75570,#75571,#75572,#75573));
#16769=EDGE_LOOP('',(#75574,#75575,#75576,#75577));
#16770=EDGE_LOOP('',(#75578,#75579,#75580,#75581,#75582,#75583));
#16771=EDGE_LOOP('',(#75584,#75585,#75586,#75587));
#16772=EDGE_LOOP('',(#75588,#75589,#75590,#75591));
#16773=EDGE_LOOP('',(#75592,#75593,#75594,#75595));
#16774=EDGE_LOOP('',(#75596,#75597,#75598,#75599));
#16775=EDGE_LOOP('',(#75600,#75601,#75602,#75603));
#16776=EDGE_LOOP('',(#75604,#75605,#75606,#75607,#75608,#75609));
#16777=EDGE_LOOP('',(#75610,#75611,#75612,#75613));
#16778=EDGE_LOOP('',(#75614,#75615,#75616,#75617));
#16779=EDGE_LOOP('',(#75618,#75619,#75620,#75621,#75622,#75623));
#16780=EDGE_LOOP('',(#75624,#75625,#75626,#75627));
#16781=EDGE_LOOP('',(#75628,#75629,#75630,#75631));
#16782=EDGE_LOOP('',(#75632,#75633,#75634,#75635));
#16783=EDGE_LOOP('',(#75636,#75637,#75638,#75639));
#16784=EDGE_LOOP('',(#75640,#75641,#75642,#75643));
#16785=EDGE_LOOP('',(#75644,#75645,#75646,#75647,#75648,#75649));
#16786=EDGE_LOOP('',(#75650,#75651,#75652,#75653));
#16787=EDGE_LOOP('',(#75654,#75655,#75656,#75657));
#16788=EDGE_LOOP('',(#75658,#75659,#75660,#75661,#75662,#75663));
#16789=EDGE_LOOP('',(#75664,#75665,#75666,#75667));
#16790=EDGE_LOOP('',(#75668,#75669,#75670,#75671));
#16791=EDGE_LOOP('',(#75672,#75673,#75674,#75675));
#16792=EDGE_LOOP('',(#75676,#75677,#75678,#75679));
#16793=EDGE_LOOP('',(#75680,#75681,#75682,#75683));
#16794=EDGE_LOOP('',(#75684,#75685,#75686,#75687,#75688,#75689));
#16795=EDGE_LOOP('',(#75690,#75691,#75692,#75693));
#16796=EDGE_LOOP('',(#75694,#75695,#75696,#75697));
#16797=EDGE_LOOP('',(#75698,#75699,#75700,#75701,#75702,#75703));
#16798=EDGE_LOOP('',(#75704,#75705,#75706,#75707));
#16799=EDGE_LOOP('',(#75708,#75709,#75710,#75711));
#16800=EDGE_LOOP('',(#75712,#75713,#75714,#75715));
#16801=EDGE_LOOP('',(#75716,#75717,#75718,#75719));
#16802=EDGE_LOOP('',(#75720,#75721,#75722,#75723));
#16803=EDGE_LOOP('',(#75724,#75725,#75726,#75727,#75728,#75729));
#16804=EDGE_LOOP('',(#75730,#75731,#75732,#75733));
#16805=EDGE_LOOP('',(#75734,#75735,#75736,#75737));
#16806=EDGE_LOOP('',(#75738,#75739,#75740,#75741,#75742,#75743));
#16807=EDGE_LOOP('',(#75744,#75745,#75746,#75747));
#16808=EDGE_LOOP('',(#75748,#75749,#75750,#75751));
#16809=EDGE_LOOP('',(#75752,#75753,#75754,#75755));
#16810=EDGE_LOOP('',(#75756,#75757,#75758,#75759));
#16811=EDGE_LOOP('',(#75760,#75761,#75762,#75763));
#16812=EDGE_LOOP('',(#75764,#75765,#75766,#75767,#75768,#75769));
#16813=EDGE_LOOP('',(#75770,#75771,#75772,#75773));
#16814=EDGE_LOOP('',(#75774,#75775,#75776,#75777));
#16815=EDGE_LOOP('',(#75778,#75779,#75780,#75781,#75782,#75783));
#16816=EDGE_LOOP('',(#75784,#75785,#75786,#75787));
#16817=EDGE_LOOP('',(#75788,#75789,#75790,#75791));
#16818=EDGE_LOOP('',(#75792,#75793,#75794,#75795));
#16819=EDGE_LOOP('',(#75796,#75797,#75798,#75799));
#16820=EDGE_LOOP('',(#75800,#75801,#75802,#75803));
#16821=EDGE_LOOP('',(#75804,#75805,#75806,#75807,#75808,#75809));
#16822=EDGE_LOOP('',(#75810,#75811,#75812,#75813));
#16823=EDGE_LOOP('',(#75814,#75815,#75816,#75817));
#16824=EDGE_LOOP('',(#75818,#75819,#75820,#75821,#75822,#75823));
#16825=EDGE_LOOP('',(#75824,#75825,#75826,#75827));
#16826=EDGE_LOOP('',(#75828,#75829,#75830,#75831));
#16827=EDGE_LOOP('',(#75832,#75833,#75834,#75835));
#16828=EDGE_LOOP('',(#75836,#75837,#75838,#75839));
#16829=EDGE_LOOP('',(#75840,#75841,#75842,#75843));
#16830=EDGE_LOOP('',(#75844,#75845,#75846,#75847,#75848,#75849));
#16831=EDGE_LOOP('',(#75850,#75851,#75852,#75853));
#16832=EDGE_LOOP('',(#75854,#75855,#75856,#75857));
#16833=EDGE_LOOP('',(#75858,#75859,#75860,#75861,#75862,#75863));
#16834=EDGE_LOOP('',(#75864,#75865,#75866,#75867));
#16835=EDGE_LOOP('',(#75868,#75869,#75870,#75871));
#16836=EDGE_LOOP('',(#75872,#75873,#75874,#75875));
#16837=EDGE_LOOP('',(#75876,#75877,#75878,#75879));
#16838=EDGE_LOOP('',(#75880,#75881,#75882,#75883));
#16839=EDGE_LOOP('',(#75884,#75885,#75886,#75887,#75888,#75889));
#16840=EDGE_LOOP('',(#75890,#75891,#75892,#75893));
#16841=EDGE_LOOP('',(#75894,#75895,#75896,#75897));
#16842=EDGE_LOOP('',(#75898,#75899,#75900,#75901,#75902,#75903));
#16843=EDGE_LOOP('',(#75904,#75905,#75906,#75907));
#16844=EDGE_LOOP('',(#75908,#75909,#75910,#75911));
#16845=EDGE_LOOP('',(#75912,#75913,#75914,#75915));
#16846=EDGE_LOOP('',(#75916,#75917,#75918,#75919));
#16847=EDGE_LOOP('',(#75920,#75921,#75922,#75923));
#16848=EDGE_LOOP('',(#75924,#75925,#75926,#75927,#75928,#75929));
#16849=EDGE_LOOP('',(#75930,#75931,#75932,#75933));
#16850=EDGE_LOOP('',(#75934,#75935,#75936,#75937));
#16851=EDGE_LOOP('',(#75938,#75939,#75940,#75941,#75942,#75943));
#16852=EDGE_LOOP('',(#75944,#75945,#75946,#75947));
#16853=EDGE_LOOP('',(#75948,#75949,#75950,#75951));
#16854=EDGE_LOOP('',(#75952,#75953,#75954,#75955));
#16855=EDGE_LOOP('',(#75956,#75957,#75958,#75959));
#16856=EDGE_LOOP('',(#75960,#75961,#75962,#75963));
#16857=EDGE_LOOP('',(#75964,#75965,#75966,#75967,#75968,#75969));
#16858=EDGE_LOOP('',(#75970,#75971,#75972,#75973));
#16859=EDGE_LOOP('',(#75974,#75975,#75976,#75977));
#16860=EDGE_LOOP('',(#75978,#75979,#75980,#75981,#75982,#75983));
#16861=EDGE_LOOP('',(#75984,#75985,#75986,#75987));
#16862=EDGE_LOOP('',(#75988,#75989,#75990,#75991));
#16863=EDGE_LOOP('',(#75992,#75993,#75994,#75995));
#16864=EDGE_LOOP('',(#75996,#75997,#75998,#75999));
#16865=EDGE_LOOP('',(#76000,#76001,#76002,#76003));
#16866=EDGE_LOOP('',(#76004,#76005,#76006,#76007,#76008,#76009));
#16867=EDGE_LOOP('',(#76010,#76011,#76012,#76013));
#16868=EDGE_LOOP('',(#76014,#76015,#76016,#76017));
#16869=EDGE_LOOP('',(#76018,#76019,#76020,#76021,#76022,#76023));
#16870=EDGE_LOOP('',(#76024,#76025,#76026,#76027));
#16871=EDGE_LOOP('',(#76028,#76029,#76030,#76031));
#16872=EDGE_LOOP('',(#76032,#76033,#76034,#76035));
#16873=EDGE_LOOP('',(#76036,#76037,#76038,#76039));
#16874=EDGE_LOOP('',(#76040,#76041,#76042,#76043));
#16875=EDGE_LOOP('',(#76044,#76045,#76046,#76047,#76048,#76049));
#16876=EDGE_LOOP('',(#76050,#76051,#76052,#76053));
#16877=EDGE_LOOP('',(#76054,#76055,#76056,#76057));
#16878=EDGE_LOOP('',(#76058,#76059,#76060,#76061,#76062,#76063));
#16879=EDGE_LOOP('',(#76064,#76065,#76066,#76067));
#16880=EDGE_LOOP('',(#76068,#76069,#76070,#76071));
#16881=EDGE_LOOP('',(#76072,#76073,#76074,#76075));
#16882=EDGE_LOOP('',(#76076,#76077,#76078,#76079));
#16883=EDGE_LOOP('',(#76080,#76081,#76082,#76083));
#16884=EDGE_LOOP('',(#76084,#76085,#76086,#76087,#76088,#76089));
#16885=EDGE_LOOP('',(#76090,#76091,#76092,#76093));
#16886=EDGE_LOOP('',(#76094,#76095,#76096,#76097));
#16887=EDGE_LOOP('',(#76098,#76099,#76100,#76101,#76102,#76103));
#16888=EDGE_LOOP('',(#76104,#76105,#76106,#76107));
#16889=EDGE_LOOP('',(#76108,#76109,#76110,#76111));
#16890=EDGE_LOOP('',(#76112,#76113,#76114,#76115));
#16891=EDGE_LOOP('',(#76116,#76117,#76118,#76119));
#16892=EDGE_LOOP('',(#76120,#76121,#76122,#76123));
#16893=EDGE_LOOP('',(#76124,#76125,#76126,#76127,#76128,#76129));
#16894=EDGE_LOOP('',(#76130,#76131,#76132,#76133));
#16895=EDGE_LOOP('',(#76134,#76135,#76136,#76137));
#16896=EDGE_LOOP('',(#76138,#76139,#76140,#76141,#76142,#76143));
#16897=EDGE_LOOP('',(#76144,#76145,#76146,#76147));
#16898=EDGE_LOOP('',(#76148,#76149,#76150,#76151));
#16899=EDGE_LOOP('',(#76152,#76153,#76154,#76155));
#16900=EDGE_LOOP('',(#76156,#76157,#76158,#76159));
#16901=EDGE_LOOP('',(#76160,#76161,#76162,#76163));
#16902=EDGE_LOOP('',(#76164,#76165,#76166,#76167,#76168,#76169));
#16903=EDGE_LOOP('',(#76170,#76171,#76172,#76173));
#16904=EDGE_LOOP('',(#76174,#76175,#76176,#76177));
#16905=EDGE_LOOP('',(#76178,#76179,#76180,#76181,#76182,#76183));
#16906=EDGE_LOOP('',(#76184,#76185,#76186,#76187));
#16907=EDGE_LOOP('',(#76188,#76189,#76190,#76191));
#16908=EDGE_LOOP('',(#76192,#76193,#76194,#76195));
#16909=EDGE_LOOP('',(#76196,#76197,#76198,#76199));
#16910=EDGE_LOOP('',(#76200,#76201,#76202,#76203));
#16911=EDGE_LOOP('',(#76204,#76205,#76206,#76207,#76208,#76209));
#16912=EDGE_LOOP('',(#76210,#76211,#76212,#76213));
#16913=EDGE_LOOP('',(#76214,#76215,#76216,#76217));
#16914=EDGE_LOOP('',(#76218,#76219,#76220,#76221,#76222,#76223));
#16915=EDGE_LOOP('',(#76224,#76225,#76226,#76227));
#16916=EDGE_LOOP('',(#76228,#76229,#76230,#76231));
#16917=EDGE_LOOP('',(#76232,#76233,#76234,#76235));
#16918=EDGE_LOOP('',(#76236,#76237,#76238,#76239));
#16919=EDGE_LOOP('',(#76240,#76241,#76242,#76243));
#16920=EDGE_LOOP('',(#76244,#76245,#76246,#76247,#76248,#76249));
#16921=EDGE_LOOP('',(#76250,#76251,#76252,#76253));
#16922=EDGE_LOOP('',(#76254,#76255,#76256,#76257));
#16923=EDGE_LOOP('',(#76258,#76259,#76260,#76261,#76262,#76263));
#16924=EDGE_LOOP('',(#76264,#76265,#76266,#76267));
#16925=EDGE_LOOP('',(#76268,#76269,#76270,#76271));
#16926=EDGE_LOOP('',(#76272,#76273,#76274,#76275));
#16927=EDGE_LOOP('',(#76276,#76277,#76278,#76279));
#16928=EDGE_LOOP('',(#76280,#76281,#76282,#76283));
#16929=EDGE_LOOP('',(#76284,#76285,#76286,#76287,#76288,#76289));
#16930=EDGE_LOOP('',(#76290,#76291,#76292,#76293));
#16931=EDGE_LOOP('',(#76294,#76295,#76296,#76297));
#16932=EDGE_LOOP('',(#76298,#76299,#76300,#76301,#76302,#76303));
#16933=EDGE_LOOP('',(#76304,#76305,#76306,#76307));
#16934=EDGE_LOOP('',(#76308,#76309,#76310,#76311));
#16935=EDGE_LOOP('',(#76312,#76313,#76314,#76315));
#16936=EDGE_LOOP('',(#76316,#76317,#76318,#76319));
#16937=EDGE_LOOP('',(#76320,#76321,#76322,#76323));
#16938=EDGE_LOOP('',(#76324,#76325,#76326,#76327,#76328,#76329));
#16939=EDGE_LOOP('',(#76330,#76331,#76332,#76333));
#16940=EDGE_LOOP('',(#76334,#76335,#76336,#76337));
#16941=EDGE_LOOP('',(#76338,#76339,#76340,#76341,#76342,#76343));
#16942=EDGE_LOOP('',(#76344,#76345,#76346,#76347));
#16943=EDGE_LOOP('',(#76348,#76349,#76350,#76351));
#16944=EDGE_LOOP('',(#76352,#76353,#76354,#76355));
#16945=EDGE_LOOP('',(#76356,#76357,#76358,#76359));
#16946=EDGE_LOOP('',(#76360,#76361,#76362,#76363));
#16947=EDGE_LOOP('',(#76364,#76365,#76366,#76367,#76368,#76369));
#16948=EDGE_LOOP('',(#76370,#76371,#76372,#76373));
#16949=EDGE_LOOP('',(#76374,#76375,#76376,#76377));
#16950=EDGE_LOOP('',(#76378,#76379,#76380,#76381,#76382,#76383));
#16951=EDGE_LOOP('',(#76384,#76385,#76386,#76387));
#16952=EDGE_LOOP('',(#76388,#76389,#76390,#76391));
#16953=EDGE_LOOP('',(#76392,#76393,#76394,#76395));
#16954=EDGE_LOOP('',(#76396,#76397,#76398,#76399));
#16955=EDGE_LOOP('',(#76400,#76401,#76402,#76403));
#16956=EDGE_LOOP('',(#76404,#76405,#76406,#76407,#76408,#76409));
#16957=EDGE_LOOP('',(#76410,#76411,#76412,#76413));
#16958=EDGE_LOOP('',(#76414,#76415,#76416,#76417));
#16959=EDGE_LOOP('',(#76418,#76419,#76420,#76421,#76422,#76423));
#16960=EDGE_LOOP('',(#76424,#76425,#76426,#76427));
#16961=EDGE_LOOP('',(#76428,#76429,#76430,#76431));
#16962=EDGE_LOOP('',(#76432,#76433,#76434,#76435));
#16963=EDGE_LOOP('',(#76436,#76437,#76438,#76439));
#16964=EDGE_LOOP('',(#76440,#76441,#76442,#76443));
#16965=EDGE_LOOP('',(#76444,#76445,#76446,#76447,#76448,#76449));
#16966=EDGE_LOOP('',(#76450,#76451,#76452,#76453));
#16967=EDGE_LOOP('',(#76454,#76455,#76456,#76457));
#16968=EDGE_LOOP('',(#76458,#76459,#76460,#76461,#76462,#76463));
#16969=EDGE_LOOP('',(#76464,#76465,#76466,#76467));
#16970=EDGE_LOOP('',(#76468,#76469,#76470,#76471));
#16971=EDGE_LOOP('',(#76472,#76473,#76474,#76475));
#16972=EDGE_LOOP('',(#76476,#76477,#76478,#76479));
#16973=EDGE_LOOP('',(#76480,#76481,#76482,#76483));
#16974=EDGE_LOOP('',(#76484,#76485,#76486,#76487,#76488,#76489));
#16975=EDGE_LOOP('',(#76490,#76491,#76492,#76493));
#16976=EDGE_LOOP('',(#76494,#76495,#76496,#76497));
#16977=EDGE_LOOP('',(#76498,#76499,#76500,#76501,#76502,#76503));
#16978=EDGE_LOOP('',(#76504,#76505,#76506,#76507));
#16979=EDGE_LOOP('',(#76508,#76509,#76510,#76511));
#16980=EDGE_LOOP('',(#76512,#76513,#76514,#76515));
#16981=EDGE_LOOP('',(#76516,#76517,#76518,#76519));
#16982=EDGE_LOOP('',(#76520,#76521,#76522,#76523));
#16983=EDGE_LOOP('',(#76524,#76525,#76526,#76527,#76528,#76529));
#16984=EDGE_LOOP('',(#76530,#76531,#76532,#76533));
#16985=EDGE_LOOP('',(#76534,#76535,#76536,#76537));
#16986=EDGE_LOOP('',(#76538,#76539,#76540,#76541,#76542,#76543));
#16987=EDGE_LOOP('',(#76544,#76545,#76546,#76547));
#16988=EDGE_LOOP('',(#76548,#76549,#76550,#76551));
#16989=EDGE_LOOP('',(#76552,#76553,#76554,#76555));
#16990=EDGE_LOOP('',(#76556,#76557,#76558,#76559));
#16991=EDGE_LOOP('',(#76560,#76561,#76562,#76563));
#16992=EDGE_LOOP('',(#76564,#76565,#76566,#76567,#76568,#76569));
#16993=EDGE_LOOP('',(#76570,#76571,#76572,#76573));
#16994=EDGE_LOOP('',(#76574,#76575,#76576,#76577));
#16995=EDGE_LOOP('',(#76578,#76579,#76580,#76581,#76582,#76583));
#16996=EDGE_LOOP('',(#76584,#76585,#76586,#76587));
#16997=EDGE_LOOP('',(#76588,#76589,#76590,#76591));
#16998=EDGE_LOOP('',(#76592,#76593,#76594,#76595));
#16999=EDGE_LOOP('',(#76596,#76597,#76598,#76599));
#17000=EDGE_LOOP('',(#76600,#76601,#76602,#76603));
#17001=EDGE_LOOP('',(#76604,#76605,#76606,#76607,#76608,#76609));
#17002=EDGE_LOOP('',(#76610,#76611,#76612,#76613));
#17003=EDGE_LOOP('',(#76614,#76615,#76616,#76617));
#17004=EDGE_LOOP('',(#76618,#76619,#76620,#76621,#76622,#76623));
#17005=EDGE_LOOP('',(#76624,#76625,#76626,#76627));
#17006=EDGE_LOOP('',(#76628,#76629,#76630,#76631));
#17007=EDGE_LOOP('',(#76632,#76633,#76634,#76635));
#17008=EDGE_LOOP('',(#76636,#76637,#76638,#76639));
#17009=EDGE_LOOP('',(#76640,#76641,#76642,#76643));
#17010=EDGE_LOOP('',(#76644));
#17011=EDGE_LOOP('',(#76645));
#17012=EDGE_LOOP('',(#76646,#76647,#76648,#76649,#76650,#76651));
#17013=EDGE_LOOP('',(#76652,#76653,#76654,#76655));
#17014=EDGE_LOOP('',(#76656,#76657,#76658,#76659));
#17015=EDGE_LOOP('',(#76660,#76661,#76662,#76663,#76664,#76665));
#17016=EDGE_LOOP('',(#76666,#76667,#76668,#76669));
#17017=EDGE_LOOP('',(#76670));
#17018=EDGE_LOOP('',(#76671));
#17019=EDGE_LOOP('',(#76672));
#17020=EDGE_LOOP('',(#76673));
#17021=EDGE_LOOP('',(#76674,#76675,#76676,#76677));
#17022=EDGE_LOOP('',(#76678,#76679,#76680,#76681));
#17023=EDGE_LOOP('',(#76682,#76683,#76684,#76685));
#17024=EDGE_LOOP('',(#76686,#76687,#76688,#76689));
#17025=EDGE_LOOP('',(#76690,#76691,#76692,#76693));
#17026=EDGE_LOOP('',(#76694,#76695,#76696,#76697,#76698,#76699,#76700,#76701,
#76702,#76703,#76704,#76705));
#17027=EDGE_LOOP('',(#76706,#76707,#76708,#76709,#76710,#76711,#76712,#76713,
#76714,#76715,#76716,#76717));
#17028=EDGE_LOOP('',(#76718,#76719,#76720,#76721));
#17029=EDGE_LOOP('',(#76722,#76723,#76724,#76725));
#17030=EDGE_LOOP('',(#76726,#76727,#76728,#76729));
#17031=EDGE_LOOP('',(#76730,#76731,#76732,#76733));
#17032=EDGE_LOOP('',(#76734,#76735,#76736,#76737,#76738));
#17033=EDGE_LOOP('',(#76739,#76740,#76741,#76742));
#17034=EDGE_LOOP('',(#76743,#76744,#76745,#76746));
#17035=EDGE_LOOP('',(#76747,#76748,#76749,#76750));
#17036=EDGE_LOOP('',(#76751,#76752,#76753,#76754));
#17037=EDGE_LOOP('',(#76755,#76756,#76757,#76758,#76759));
#17038=EDGE_LOOP('',(#76760,#76761,#76762,#76763));
#17039=EDGE_LOOP('',(#76764,#76765,#76766,#76767));
#17040=EDGE_LOOP('',(#76768,#76769,#76770,#76771));
#17041=EDGE_LOOP('',(#76772,#76773,#76774,#76775));
#17042=EDGE_LOOP('',(#76776,#76777,#76778,#76779));
#17043=EDGE_LOOP('',(#76780,#76781,#76782,#76783));
#17044=EDGE_LOOP('',(#76784,#76785,#76786,#76787));
#17045=EDGE_LOOP('',(#76788,#76789,#76790,#76791));
#17046=EDGE_LOOP('',(#76792,#76793,#76794,#76795));
#17047=EDGE_LOOP('',(#76796,#76797,#76798,#76799,#76800));
#17048=EDGE_LOOP('',(#76801,#76802,#76803,#76804,#76805));
#17049=EDGE_LOOP('',(#76806,#76807,#76808,#76809));
#17050=EDGE_LOOP('',(#76810,#76811,#76812,#76813));
#17051=EDGE_LOOP('',(#76814,#76815,#76816,#76817));
#17052=EDGE_LOOP('',(#76818,#76819,#76820,#76821));
#17053=EDGE_LOOP('',(#76822,#76823,#76824,#76825));
#17054=EDGE_LOOP('',(#76826,#76827,#76828,#76829));
#17055=EDGE_LOOP('',(#76830,#76831,#76832,#76833));
#17056=EDGE_LOOP('',(#76834,#76835,#76836,#76837));
#17057=EDGE_LOOP('',(#76838,#76839,#76840,#76841,#76842));
#17058=EDGE_LOOP('',(#76843,#76844,#76845,#76846));
#17059=EDGE_LOOP('',(#76847,#76848,#76849,#76850,#76851,#76852,#76853,#76854,
#76855,#76856,#76857,#76858));
#17060=EDGE_LOOP('',(#76859,#76860,#76861,#76862,#76863,#76864,#76865,#76866,
#76867,#76868,#76869,#76870));
#17061=EDGE_LOOP('',(#76871,#76872,#76873,#76874));
#17062=EDGE_LOOP('',(#76875,#76876,#76877,#76878,#76879,#76880,#76881,#76882,
#76883,#76884,#76885,#76886));
#17063=EDGE_LOOP('',(#76887,#76888,#76889,#76890,#76891,#76892,#76893,#76894,
#76895,#76896,#76897,#76898));
#17064=EDGE_LOOP('',(#76899,#76900,#76901,#76902));
#17065=EDGE_LOOP('',(#76903,#76904,#76905,#76906,#76907,#76908,#76909,#76910,
#76911,#76912,#76913,#76914));
#17066=EDGE_LOOP('',(#76915,#76916,#76917,#76918,#76919,#76920,#76921,#76922,
#76923,#76924,#76925,#76926));
#17067=EDGE_LOOP('',(#76927,#76928,#76929,#76930));
#17068=EDGE_LOOP('',(#76931,#76932,#76933,#76934,#76935,#76936,#76937,#76938,
#76939,#76940,#76941,#76942));
#17069=EDGE_LOOP('',(#76943,#76944,#76945,#76946,#76947,#76948,#76949,#76950,
#76951,#76952,#76953,#76954));
#17070=EDGE_LOOP('',(#76955,#76956,#76957,#76958));
#17071=EDGE_LOOP('',(#76959,#76960,#76961,#76962,#76963,#76964,#76965,#76966,
#76967,#76968,#76969,#76970));
#17072=EDGE_LOOP('',(#76971,#76972,#76973,#76974,#76975,#76976,#76977,#76978,
#76979,#76980,#76981,#76982));
#17073=EDGE_LOOP('',(#76983,#76984,#76985,#76986));
#17074=EDGE_LOOP('',(#76987,#76988,#76989,#76990,#76991,#76992,#76993,#76994,
#76995,#76996,#76997,#76998));
#17075=EDGE_LOOP('',(#76999,#77000,#77001,#77002,#77003,#77004,#77005,#77006,
#77007,#77008,#77009,#77010));
#17076=EDGE_LOOP('',(#77011,#77012,#77013,#77014));
#17077=EDGE_LOOP('',(#77015,#77016,#77017,#77018,#77019,#77020,#77021,#77022,
#77023,#77024,#77025,#77026));
#17078=EDGE_LOOP('',(#77027,#77028,#77029,#77030,#77031,#77032,#77033,#77034,
#77035,#77036,#77037,#77038));
#17079=EDGE_LOOP('',(#77039,#77040,#77041,#77042));
#17080=EDGE_LOOP('',(#77043,#77044,#77045,#77046,#77047,#77048,#77049,#77050,
#77051,#77052,#77053,#77054));
#17081=EDGE_LOOP('',(#77055,#77056,#77057,#77058,#77059,#77060,#77061,#77062,
#77063,#77064,#77065,#77066));
#17082=EDGE_LOOP('',(#77067,#77068,#77069,#77070));
#17083=EDGE_LOOP('',(#77071,#77072,#77073,#77074,#77075,#77076,#77077,#77078,
#77079,#77080,#77081,#77082));
#17084=EDGE_LOOP('',(#77083,#77084,#77085,#77086,#77087,#77088,#77089,#77090,
#77091,#77092,#77093,#77094));
#17085=EDGE_LOOP('',(#77095,#77096,#77097,#77098));
#17086=EDGE_LOOP('',(#77099,#77100,#77101,#77102,#77103,#77104,#77105,#77106,
#77107,#77108,#77109,#77110));
#17087=EDGE_LOOP('',(#77111,#77112,#77113,#77114,#77115,#77116,#77117,#77118,
#77119,#77120,#77121,#77122));
#17088=EDGE_LOOP('',(#77123,#77124,#77125,#77126));
#17089=EDGE_LOOP('',(#77127,#77128,#77129,#77130,#77131,#77132,#77133,#77134,
#77135,#77136,#77137,#77138));
#17090=EDGE_LOOP('',(#77139,#77140,#77141,#77142,#77143,#77144,#77145,#77146,
#77147,#77148,#77149,#77150));
#17091=EDGE_LOOP('',(#77151,#77152,#77153,#77154));
#17092=EDGE_LOOP('',(#77155,#77156,#77157,#77158,#77159,#77160,#77161,#77162,
#77163,#77164,#77165,#77166));
#17093=EDGE_LOOP('',(#77167,#77168,#77169,#77170,#77171,#77172,#77173,#77174,
#77175,#77176,#77177,#77178));
#17094=EDGE_LOOP('',(#77179,#77180,#77181,#77182));
#17095=EDGE_LOOP('',(#77183,#77184,#77185,#77186,#77187,#77188,#77189,#77190,
#77191,#77192,#77193,#77194));
#17096=EDGE_LOOP('',(#77195,#77196,#77197,#77198,#77199,#77200,#77201,#77202,
#77203,#77204,#77205,#77206));
#17097=EDGE_LOOP('',(#77207,#77208,#77209,#77210));
#17098=EDGE_LOOP('',(#77211,#77212,#77213,#77214,#77215,#77216,#77217,#77218,
#77219,#77220,#77221,#77222));
#17099=EDGE_LOOP('',(#77223,#77224,#77225,#77226,#77227,#77228,#77229,#77230,
#77231,#77232,#77233,#77234));
#17100=EDGE_LOOP('',(#77235,#77236,#77237,#77238));
#17101=EDGE_LOOP('',(#77239,#77240,#77241,#77242,#77243,#77244,#77245,#77246,
#77247,#77248,#77249,#77250));
#17102=EDGE_LOOP('',(#77251,#77252,#77253,#77254,#77255,#77256,#77257,#77258,
#77259,#77260,#77261,#77262));
#17103=EDGE_LOOP('',(#77263,#77264,#77265,#77266));
#17104=EDGE_LOOP('',(#77267,#77268,#77269,#77270,#77271,#77272,#77273,#77274,
#77275,#77276,#77277,#77278));
#17105=EDGE_LOOP('',(#77279,#77280,#77281,#77282,#77283,#77284,#77285,#77286,
#77287,#77288,#77289,#77290));
#17106=EDGE_LOOP('',(#77291,#77292,#77293,#77294));
#17107=EDGE_LOOP('',(#77295,#77296,#77297,#77298,#77299,#77300,#77301,#77302,
#77303,#77304,#77305,#77306));
#17108=EDGE_LOOP('',(#77307,#77308,#77309,#77310,#77311,#77312,#77313,#77314,
#77315,#77316,#77317,#77318));
#17109=EDGE_LOOP('',(#77319,#77320,#77321,#77322));
#17110=EDGE_LOOP('',(#77323,#77324,#77325,#77326,#77327,#77328,#77329,#77330,
#77331,#77332,#77333,#77334));
#17111=EDGE_LOOP('',(#77335,#77336,#77337,#77338,#77339,#77340,#77341,#77342,
#77343,#77344,#77345,#77346));
#17112=EDGE_LOOP('',(#77347,#77348,#77349,#77350));
#17113=EDGE_LOOP('',(#77351,#77352,#77353,#77354,#77355,#77356,#77357,#77358,
#77359,#77360,#77361,#77362));
#17114=EDGE_LOOP('',(#77363,#77364,#77365,#77366,#77367,#77368,#77369,#77370,
#77371,#77372,#77373,#77374));
#17115=EDGE_LOOP('',(#77375,#77376,#77377,#77378));
#17116=EDGE_LOOP('',(#77379,#77380,#77381,#77382,#77383,#77384,#77385,#77386,
#77387,#77388,#77389,#77390));
#17117=EDGE_LOOP('',(#77391,#77392,#77393,#77394,#77395,#77396,#77397,#77398,
#77399,#77400,#77401,#77402));
#17118=EDGE_LOOP('',(#77403,#77404,#77405,#77406));
#17119=EDGE_LOOP('',(#77407,#77408,#77409,#77410,#77411,#77412,#77413,#77414,
#77415,#77416,#77417,#77418));
#17120=EDGE_LOOP('',(#77419,#77420,#77421,#77422,#77423,#77424,#77425,#77426,
#77427,#77428,#77429,#77430));
#17121=EDGE_LOOP('',(#77431,#77432,#77433,#77434));
#17122=EDGE_LOOP('',(#77435,#77436,#77437,#77438,#77439,#77440,#77441,#77442,
#77443,#77444,#77445,#77446));
#17123=EDGE_LOOP('',(#77447,#77448,#77449,#77450,#77451,#77452,#77453,#77454,
#77455,#77456,#77457,#77458));
#17124=EDGE_LOOP('',(#77459,#77460,#77461,#77462));
#17125=EDGE_LOOP('',(#77463,#77464,#77465,#77466,#77467,#77468,#77469,#77470,
#77471,#77472,#77473,#77474));
#17126=EDGE_LOOP('',(#77475,#77476,#77477,#77478,#77479,#77480,#77481,#77482,
#77483,#77484,#77485,#77486));
#17127=EDGE_LOOP('',(#77487,#77488,#77489,#77490));
#17128=EDGE_LOOP('',(#77491,#77492,#77493,#77494,#77495,#77496,#77497,#77498,
#77499,#77500,#77501,#77502));
#17129=EDGE_LOOP('',(#77503,#77504,#77505,#77506,#77507,#77508,#77509,#77510,
#77511,#77512,#77513,#77514));
#17130=EDGE_LOOP('',(#77515,#77516,#77517,#77518));
#17131=EDGE_LOOP('',(#77519,#77520,#77521,#77522,#77523,#77524,#77525,#77526,
#77527,#77528,#77529,#77530));
#17132=EDGE_LOOP('',(#77531,#77532,#77533,#77534,#77535,#77536,#77537,#77538,
#77539,#77540,#77541,#77542));
#17133=EDGE_LOOP('',(#77543,#77544,#77545,#77546));
#17134=EDGE_LOOP('',(#77547,#77548,#77549,#77550,#77551,#77552,#77553,#77554,
#77555,#77556,#77557,#77558));
#17135=EDGE_LOOP('',(#77559,#77560,#77561,#77562,#77563,#77564,#77565,#77566,
#77567,#77568,#77569,#77570));
#17136=EDGE_LOOP('',(#77571,#77572,#77573,#77574));
#17137=EDGE_LOOP('',(#77575,#77576,#77577,#77578,#77579,#77580,#77581,#77582,
#77583,#77584,#77585,#77586));
#17138=EDGE_LOOP('',(#77587,#77588,#77589,#77590,#77591,#77592,#77593,#77594,
#77595,#77596,#77597,#77598));
#17139=EDGE_LOOP('',(#77599,#77600,#77601,#77602));
#17140=EDGE_LOOP('',(#77603,#77604,#77605,#77606,#77607,#77608,#77609,#77610,
#77611,#77612,#77613,#77614));
#17141=EDGE_LOOP('',(#77615,#77616,#77617,#77618,#77619,#77620,#77621,#77622,
#77623,#77624,#77625,#77626));
#17142=EDGE_LOOP('',(#77627,#77628,#77629,#77630));
#17143=EDGE_LOOP('',(#77631,#77632,#77633,#77634,#77635,#77636,#77637,#77638,
#77639,#77640,#77641,#77642));
#17144=EDGE_LOOP('',(#77643,#77644,#77645,#77646,#77647,#77648,#77649,#77650,
#77651,#77652,#77653,#77654));
#17145=EDGE_LOOP('',(#77655,#77656,#77657,#77658));
#17146=EDGE_LOOP('',(#77659,#77660,#77661,#77662,#77663,#77664,#77665,#77666,
#77667,#77668,#77669,#77670));
#17147=EDGE_LOOP('',(#77671,#77672,#77673,#77674,#77675,#77676,#77677,#77678,
#77679,#77680,#77681,#77682));
#17148=EDGE_LOOP('',(#77683,#77684,#77685,#77686));
#17149=EDGE_LOOP('',(#77687,#77688,#77689,#77690,#77691,#77692,#77693,#77694,
#77695,#77696,#77697,#77698));
#17150=EDGE_LOOP('',(#77699,#77700,#77701,#77702,#77703,#77704,#77705,#77706,
#77707,#77708,#77709,#77710));
#17151=EDGE_LOOP('',(#77711,#77712,#77713,#77714));
#17152=EDGE_LOOP('',(#77715,#77716,#77717,#77718,#77719,#77720,#77721,#77722,
#77723,#77724,#77725,#77726));
#17153=EDGE_LOOP('',(#77727,#77728,#77729,#77730,#77731,#77732,#77733,#77734,
#77735,#77736,#77737,#77738));
#17154=EDGE_LOOP('',(#77739,#77740,#77741,#77742));
#17155=EDGE_LOOP('',(#77743,#77744,#77745,#77746,#77747,#77748,#77749,#77750,
#77751,#77752,#77753,#77754));
#17156=EDGE_LOOP('',(#77755,#77756,#77757,#77758,#77759,#77760,#77761,#77762,
#77763,#77764,#77765,#77766));
#17157=EDGE_LOOP('',(#77767,#77768,#77769,#77770));
#17158=EDGE_LOOP('',(#77771,#77772,#77773,#77774,#77775,#77776,#77777,#77778,
#77779,#77780,#77781,#77782));
#17159=EDGE_LOOP('',(#77783,#77784,#77785,#77786,#77787,#77788,#77789,#77790,
#77791,#77792,#77793,#77794));
#17160=EDGE_LOOP('',(#77795,#77796,#77797,#77798));
#17161=EDGE_LOOP('',(#77799,#77800,#77801,#77802,#77803,#77804,#77805,#77806,
#77807,#77808,#77809,#77810));
#17162=EDGE_LOOP('',(#77811,#77812,#77813,#77814,#77815,#77816,#77817,#77818,
#77819,#77820,#77821,#77822));
#17163=EDGE_LOOP('',(#77823,#77824,#77825,#77826));
#17164=EDGE_LOOP('',(#77827,#77828,#77829,#77830,#77831,#77832,#77833,#77834,
#77835,#77836,#77837,#77838));
#17165=EDGE_LOOP('',(#77839,#77840,#77841,#77842,#77843,#77844,#77845,#77846,
#77847,#77848,#77849,#77850));
#17166=EDGE_LOOP('',(#77851,#77852,#77853,#77854));
#17167=EDGE_LOOP('',(#77855,#77856,#77857,#77858,#77859,#77860,#77861,#77862,
#77863,#77864,#77865,#77866));
#17168=EDGE_LOOP('',(#77867,#77868,#77869,#77870,#77871,#77872,#77873,#77874,
#77875,#77876,#77877,#77878));
#17169=EDGE_LOOP('',(#77879,#77880,#77881,#77882));
#17170=EDGE_LOOP('',(#77883,#77884,#77885,#77886,#77887,#77888,#77889,#77890,
#77891,#77892,#77893,#77894));
#17171=EDGE_LOOP('',(#77895,#77896,#77897,#77898,#77899,#77900,#77901,#77902,
#77903,#77904,#77905,#77906));
#17172=EDGE_LOOP('',(#77907,#77908,#77909,#77910));
#17173=EDGE_LOOP('',(#77911,#77912,#77913,#77914,#77915,#77916,#77917,#77918,
#77919,#77920,#77921,#77922));
#17174=EDGE_LOOP('',(#77923,#77924,#77925,#77926,#77927,#77928,#77929,#77930,
#77931,#77932,#77933,#77934));
#17175=EDGE_LOOP('',(#77935,#77936,#77937,#77938));
#17176=EDGE_LOOP('',(#77939,#77940,#77941,#77942,#77943,#77944,#77945,#77946,
#77947,#77948,#77949,#77950));
#17177=EDGE_LOOP('',(#77951,#77952,#77953,#77954,#77955,#77956,#77957,#77958,
#77959,#77960,#77961,#77962));
#17178=EDGE_LOOP('',(#77963,#77964,#77965,#77966));
#17179=EDGE_LOOP('',(#77967,#77968,#77969,#77970,#77971,#77972,#77973,#77974,
#77975,#77976,#77977,#77978));
#17180=EDGE_LOOP('',(#77979,#77980,#77981,#77982,#77983,#77984,#77985,#77986,
#77987,#77988,#77989,#77990));
#17181=EDGE_LOOP('',(#77991,#77992,#77993,#77994));
#17182=EDGE_LOOP('',(#77995,#77996,#77997,#77998,#77999,#78000,#78001,#78002,
#78003,#78004,#78005,#78006));
#17183=EDGE_LOOP('',(#78007,#78008,#78009,#78010,#78011,#78012,#78013,#78014,
#78015,#78016,#78017,#78018));
#17184=EDGE_LOOP('',(#78019,#78020,#78021,#78022));
#17185=EDGE_LOOP('',(#78023,#78024,#78025,#78026,#78027,#78028,#78029,#78030,
#78031,#78032,#78033,#78034));
#17186=EDGE_LOOP('',(#78035,#78036,#78037,#78038,#78039,#78040,#78041,#78042,
#78043,#78044,#78045,#78046));
#17187=EDGE_LOOP('',(#78047,#78048,#78049,#78050));
#17188=EDGE_LOOP('',(#78051,#78052,#78053,#78054,#78055,#78056,#78057,#78058,
#78059,#78060,#78061,#78062));
#17189=EDGE_LOOP('',(#78063,#78064,#78065,#78066,#78067,#78068,#78069,#78070,
#78071,#78072,#78073,#78074));
#17190=EDGE_LOOP('',(#78075,#78076,#78077,#78078));
#17191=EDGE_LOOP('',(#78079,#78080,#78081,#78082,#78083,#78084,#78085,#78086,
#78087,#78088,#78089,#78090));
#17192=EDGE_LOOP('',(#78091,#78092,#78093,#78094,#78095,#78096,#78097,#78098,
#78099,#78100,#78101,#78102));
#17193=EDGE_LOOP('',(#78103,#78104,#78105,#78106));
#17194=EDGE_LOOP('',(#78107,#78108,#78109,#78110,#78111,#78112,#78113,#78114,
#78115,#78116,#78117,#78118));
#17195=EDGE_LOOP('',(#78119,#78120,#78121,#78122,#78123,#78124,#78125,#78126,
#78127,#78128,#78129,#78130));
#17196=EDGE_LOOP('',(#78131,#78132,#78133,#78134));
#17197=EDGE_LOOP('',(#78135,#78136,#78137,#78138,#78139,#78140,#78141,#78142,
#78143,#78144,#78145,#78146));
#17198=EDGE_LOOP('',(#78147,#78148,#78149,#78150,#78151,#78152,#78153,#78154,
#78155,#78156,#78157,#78158));
#17199=EDGE_LOOP('',(#78159,#78160,#78161,#78162));
#17200=EDGE_LOOP('',(#78163,#78164,#78165,#78166,#78167,#78168,#78169,#78170,
#78171,#78172,#78173,#78174));
#17201=EDGE_LOOP('',(#78175,#78176,#78177,#78178,#78179,#78180,#78181,#78182,
#78183,#78184,#78185,#78186));
#17202=EDGE_LOOP('',(#78187,#78188,#78189,#78190));
#17203=EDGE_LOOP('',(#78191,#78192,#78193,#78194,#78195,#78196,#78197,#78198,
#78199,#78200,#78201,#78202));
#17204=EDGE_LOOP('',(#78203,#78204,#78205,#78206,#78207,#78208,#78209,#78210,
#78211,#78212,#78213,#78214));
#17205=EDGE_LOOP('',(#78215,#78216,#78217,#78218));
#17206=EDGE_LOOP('',(#78219,#78220,#78221,#78222,#78223,#78224,#78225,#78226,
#78227,#78228,#78229,#78230));
#17207=EDGE_LOOP('',(#78231,#78232,#78233,#78234,#78235,#78236,#78237,#78238,
#78239,#78240,#78241,#78242));
#17208=EDGE_LOOP('',(#78243,#78244,#78245,#78246));
#17209=EDGE_LOOP('',(#78247,#78248,#78249,#78250,#78251,#78252,#78253,#78254,
#78255,#78256,#78257,#78258));
#17210=EDGE_LOOP('',(#78259,#78260,#78261,#78262,#78263,#78264,#78265,#78266,
#78267,#78268,#78269,#78270));
#17211=EDGE_LOOP('',(#78271,#78272,#78273,#78274));
#17212=EDGE_LOOP('',(#78275,#78276,#78277,#78278,#78279,#78280,#78281,#78282,
#78283,#78284,#78285,#78286));
#17213=EDGE_LOOP('',(#78287,#78288,#78289,#78290,#78291,#78292,#78293,#78294,
#78295,#78296,#78297,#78298));
#17214=EDGE_LOOP('',(#78299,#78300,#78301,#78302));
#17215=EDGE_LOOP('',(#78303,#78304,#78305,#78306,#78307,#78308,#78309,#78310,
#78311,#78312,#78313,#78314));
#17216=EDGE_LOOP('',(#78315,#78316,#78317,#78318,#78319,#78320,#78321,#78322,
#78323,#78324,#78325,#78326));
#17217=EDGE_LOOP('',(#78327,#78328,#78329,#78330));
#17218=EDGE_LOOP('',(#78331,#78332,#78333,#78334,#78335,#78336,#78337,#78338,
#78339,#78340,#78341,#78342));
#17219=EDGE_LOOP('',(#78343,#78344,#78345,#78346,#78347,#78348,#78349,#78350,
#78351,#78352,#78353,#78354));
#17220=EDGE_LOOP('',(#78355,#78356,#78357,#78358));
#17221=EDGE_LOOP('',(#78359,#78360,#78361,#78362,#78363,#78364,#78365,#78366,
#78367,#78368,#78369,#78370));
#17222=EDGE_LOOP('',(#78371,#78372,#78373,#78374,#78375,#78376,#78377,#78378,
#78379,#78380,#78381,#78382));
#17223=EDGE_LOOP('',(#78383,#78384,#78385,#78386));
#17224=EDGE_LOOP('',(#78387,#78388,#78389,#78390,#78391,#78392,#78393,#78394,
#78395,#78396,#78397,#78398));
#17225=EDGE_LOOP('',(#78399,#78400,#78401,#78402,#78403,#78404,#78405,#78406,
#78407,#78408,#78409,#78410));
#17226=EDGE_LOOP('',(#78411,#78412,#78413,#78414));
#17227=EDGE_LOOP('',(#78415,#78416,#78417,#78418,#78419,#78420,#78421,#78422,
#78423,#78424,#78425,#78426));
#17228=EDGE_LOOP('',(#78427,#78428,#78429,#78430,#78431,#78432,#78433,#78434,
#78435,#78436,#78437,#78438));
#17229=EDGE_LOOP('',(#78439,#78440,#78441,#78442));
#17230=EDGE_LOOP('',(#78443,#78444,#78445,#78446,#78447,#78448,#78449,#78450,
#78451,#78452,#78453,#78454));
#17231=EDGE_LOOP('',(#78455,#78456,#78457,#78458,#78459,#78460,#78461,#78462,
#78463,#78464,#78465,#78466));
#17232=EDGE_LOOP('',(#78467,#78468,#78469,#78470));
#17233=EDGE_LOOP('',(#78471,#78472,#78473,#78474,#78475,#78476,#78477,#78478,
#78479,#78480,#78481,#78482));
#17234=EDGE_LOOP('',(#78483,#78484,#78485,#78486,#78487,#78488,#78489,#78490,
#78491,#78492,#78493,#78494));
#17235=EDGE_LOOP('',(#78495,#78496,#78497,#78498));
#17236=EDGE_LOOP('',(#78499,#78500,#78501,#78502));
#17237=EDGE_LOOP('',(#78503,#78504,#78505,#78506));
#17238=EDGE_LOOP('',(#78507,#78508,#78509,#78510));
#17239=EDGE_LOOP('',(#78511,#78512,#78513,#78514));
#17240=EDGE_LOOP('',(#78515,#78516,#78517,#78518));
#17241=EDGE_LOOP('',(#78519,#78520,#78521,#78522));
#17242=EDGE_LOOP('',(#78523,#78524,#78525,#78526));
#17243=EDGE_LOOP('',(#78527,#78528,#78529,#78530));
#17244=EDGE_LOOP('',(#78531,#78532,#78533,#78534));
#17245=EDGE_LOOP('',(#78535,#78536,#78537,#78538));
#17246=EDGE_LOOP('',(#78539,#78540,#78541,#78542));
#17247=EDGE_LOOP('',(#78543,#78544,#78545,#78546));
#17248=EDGE_LOOP('',(#78547,#78548,#78549,#78550));
#17249=EDGE_LOOP('',(#78551,#78552,#78553,#78554));
#17250=EDGE_LOOP('',(#78555,#78556,#78557,#78558));
#17251=EDGE_LOOP('',(#78559,#78560,#78561,#78562));
#17252=EDGE_LOOP('',(#78563,#78564,#78565,#78566));
#17253=EDGE_LOOP('',(#78567,#78568,#78569,#78570));
#17254=EDGE_LOOP('',(#78571,#78572,#78573,#78574));
#17255=EDGE_LOOP('',(#78575,#78576,#78577,#78578));
#17256=EDGE_LOOP('',(#78579,#78580,#78581,#78582));
#17257=EDGE_LOOP('',(#78583,#78584,#78585,#78586));
#17258=EDGE_LOOP('',(#78587,#78588,#78589,#78590));
#17259=EDGE_LOOP('',(#78591,#78592,#78593,#78594));
#17260=EDGE_LOOP('',(#78595,#78596,#78597,#78598));
#17261=EDGE_LOOP('',(#78599,#78600,#78601,#78602));
#17262=EDGE_LOOP('',(#78603,#78604,#78605,#78606));
#17263=EDGE_LOOP('',(#78607,#78608,#78609,#78610));
#17264=EDGE_LOOP('',(#78611,#78612,#78613,#78614));
#17265=EDGE_LOOP('',(#78615,#78616,#78617,#78618));
#17266=EDGE_LOOP('',(#78619,#78620,#78621,#78622));
#17267=EDGE_LOOP('',(#78623,#78624,#78625,#78626));
#17268=EDGE_LOOP('',(#78627,#78628,#78629,#78630));
#17269=EDGE_LOOP('',(#78631,#78632,#78633,#78634));
#17270=EDGE_LOOP('',(#78635,#78636,#78637,#78638));
#17271=EDGE_LOOP('',(#78639,#78640,#78641,#78642));
#17272=EDGE_LOOP('',(#78643,#78644,#78645,#78646));
#17273=EDGE_LOOP('',(#78647,#78648,#78649,#78650));
#17274=EDGE_LOOP('',(#78651,#78652,#78653,#78654));
#17275=EDGE_LOOP('',(#78655,#78656,#78657,#78658));
#17276=EDGE_LOOP('',(#78659,#78660,#78661,#78662));
#17277=EDGE_LOOP('',(#78663,#78664,#78665,#78666));
#17278=EDGE_LOOP('',(#78667,#78668,#78669,#78670));
#17279=EDGE_LOOP('',(#78671,#78672,#78673,#78674));
#17280=EDGE_LOOP('',(#78675,#78676,#78677,#78678));
#17281=EDGE_LOOP('',(#78679,#78680,#78681,#78682));
#17282=EDGE_LOOP('',(#78683,#78684,#78685,#78686));
#17283=EDGE_LOOP('',(#78687,#78688,#78689,#78690));
#17284=EDGE_LOOP('',(#78691,#78692,#78693,#78694));
#17285=EDGE_LOOP('',(#78695,#78696,#78697,#78698));
#17286=EDGE_LOOP('',(#78699,#78700,#78701,#78702));
#17287=EDGE_LOOP('',(#78703,#78704,#78705,#78706));
#17288=EDGE_LOOP('',(#78707,#78708,#78709,#78710));
#17289=EDGE_LOOP('',(#78711,#78712,#78713,#78714));
#17290=EDGE_LOOP('',(#78715,#78716,#78717,#78718));
#17291=EDGE_LOOP('',(#78719,#78720,#78721,#78722));
#17292=EDGE_LOOP('',(#78723,#78724,#78725,#78726));
#17293=EDGE_LOOP('',(#78727,#78728,#78729,#78730));
#17294=EDGE_LOOP('',(#78731,#78732,#78733,#78734));
#17295=EDGE_LOOP('',(#78735,#78736,#78737,#78738));
#17296=EDGE_LOOP('',(#78739,#78740,#78741,#78742));
#17297=EDGE_LOOP('',(#78743,#78744,#78745,#78746));
#17298=EDGE_LOOP('',(#78747,#78748,#78749,#78750));
#17299=EDGE_LOOP('',(#78751,#78752,#78753,#78754));
#17300=EDGE_LOOP('',(#78755,#78756,#78757,#78758));
#17301=EDGE_LOOP('',(#78759,#78760,#78761,#78762));
#17302=EDGE_LOOP('',(#78763,#78764,#78765,#78766));
#17303=EDGE_LOOP('',(#78767,#78768,#78769,#78770));
#17304=EDGE_LOOP('',(#78771,#78772,#78773,#78774));
#17305=EDGE_LOOP('',(#78775,#78776,#78777,#78778));
#17306=EDGE_LOOP('',(#78779,#78780,#78781,#78782));
#17307=EDGE_LOOP('',(#78783,#78784,#78785,#78786));
#17308=EDGE_LOOP('',(#78787,#78788,#78789,#78790));
#17309=EDGE_LOOP('',(#78791,#78792,#78793,#78794));
#17310=EDGE_LOOP('',(#78795,#78796,#78797,#78798));
#17311=EDGE_LOOP('',(#78799,#78800,#78801,#78802));
#17312=EDGE_LOOP('',(#78803,#78804,#78805,#78806));
#17313=EDGE_LOOP('',(#78807,#78808,#78809,#78810));
#17314=EDGE_LOOP('',(#78811,#78812,#78813,#78814));
#17315=EDGE_LOOP('',(#78815,#78816,#78817,#78818));
#17316=EDGE_LOOP('',(#78819,#78820,#78821,#78822));
#17317=EDGE_LOOP('',(#78823,#78824,#78825,#78826));
#17318=EDGE_LOOP('',(#78827,#78828,#78829,#78830));
#17319=EDGE_LOOP('',(#78831,#78832,#78833,#78834));
#17320=EDGE_LOOP('',(#78835,#78836,#78837,#78838));
#17321=EDGE_LOOP('',(#78839,#78840,#78841,#78842));
#17322=EDGE_LOOP('',(#78843,#78844,#78845,#78846));
#17323=EDGE_LOOP('',(#78847,#78848,#78849,#78850));
#17324=EDGE_LOOP('',(#78851,#78852,#78853,#78854));
#17325=EDGE_LOOP('',(#78855,#78856,#78857,#78858));
#17326=EDGE_LOOP('',(#78859,#78860,#78861,#78862));
#17327=EDGE_LOOP('',(#78863,#78864,#78865,#78866));
#17328=EDGE_LOOP('',(#78867,#78868,#78869,#78870));
#17329=EDGE_LOOP('',(#78871,#78872,#78873,#78874));
#17330=EDGE_LOOP('',(#78875,#78876,#78877,#78878));
#17331=EDGE_LOOP('',(#78879,#78880,#78881,#78882));
#17332=EDGE_LOOP('',(#78883,#78884,#78885,#78886));
#17333=EDGE_LOOP('',(#78887,#78888,#78889,#78890));
#17334=EDGE_LOOP('',(#78891,#78892,#78893,#78894));
#17335=EDGE_LOOP('',(#78895,#78896,#78897,#78898));
#17336=EDGE_LOOP('',(#78899,#78900,#78901,#78902));
#17337=EDGE_LOOP('',(#78903,#78904,#78905,#78906));
#17338=EDGE_LOOP('',(#78907,#78908,#78909,#78910));
#17339=EDGE_LOOP('',(#78911,#78912,#78913,#78914));
#17340=EDGE_LOOP('',(#78915,#78916,#78917,#78918));
#17341=EDGE_LOOP('',(#78919,#78920,#78921,#78922));
#17342=EDGE_LOOP('',(#78923,#78924,#78925,#78926));
#17343=EDGE_LOOP('',(#78927,#78928,#78929,#78930));
#17344=EDGE_LOOP('',(#78931,#78932,#78933,#78934));
#17345=EDGE_LOOP('',(#78935,#78936,#78937,#78938));
#17346=EDGE_LOOP('',(#78939,#78940,#78941,#78942));
#17347=EDGE_LOOP('',(#78943,#78944,#78945,#78946));
#17348=EDGE_LOOP('',(#78947,#78948,#78949,#78950));
#17349=EDGE_LOOP('',(#78951,#78952,#78953,#78954));
#17350=EDGE_LOOP('',(#78955,#78956,#78957,#78958));
#17351=EDGE_LOOP('',(#78959,#78960,#78961,#78962));
#17352=EDGE_LOOP('',(#78963,#78964,#78965,#78966));
#17353=EDGE_LOOP('',(#78967,#78968,#78969,#78970));
#17354=EDGE_LOOP('',(#78971,#78972,#78973,#78974));
#17355=EDGE_LOOP('',(#78975,#78976,#78977,#78978,#78979));
#17356=EDGE_LOOP('',(#78980,#78981,#78982,#78983));
#17357=EDGE_LOOP('',(#78984,#78985,#78986,#78987));
#17358=EDGE_LOOP('',(#78988,#78989,#78990,#78991));
#17359=EDGE_LOOP('',(#78992,#78993,#78994,#78995));
#17360=EDGE_LOOP('',(#78996,#78997,#78998,#78999,#79000));
#17361=EDGE_LOOP('',(#79001,#79002,#79003,#79004));
#17362=EDGE_LOOP('',(#79005,#79006,#79007,#79008));
#17363=EDGE_LOOP('',(#79009,#79010,#79011,#79012));
#17364=EDGE_LOOP('',(#79013,#79014,#79015,#79016));
#17365=EDGE_LOOP('',(#79017,#79018,#79019,#79020));
#17366=EDGE_LOOP('',(#79021,#79022,#79023,#79024));
#17367=EDGE_LOOP('',(#79025,#79026,#79027,#79028));
#17368=EDGE_LOOP('',(#79029,#79030,#79031,#79032));
#17369=EDGE_LOOP('',(#79033,#79034,#79035,#79036));
#17370=EDGE_LOOP('',(#79037,#79038,#79039,#79040));
#17371=EDGE_LOOP('',(#79041,#79042,#79043,#79044,#79045));
#17372=EDGE_LOOP('',(#79046,#79047,#79048,#79049));
#17373=EDGE_LOOP('',(#79050,#79051,#79052,#79053));
#17374=EDGE_LOOP('',(#79054,#79055,#79056,#79057));
#17375=EDGE_LOOP('',(#79058,#79059,#79060,#79061));
#17376=EDGE_LOOP('',(#79062,#79063,#79064,#79065));
#17377=EDGE_LOOP('',(#79066,#79067,#79068,#79069));
#17378=EDGE_LOOP('',(#79070,#79071,#79072,#79073));
#17379=EDGE_LOOP('',(#79074,#79075,#79076,#79077));
#17380=EDGE_LOOP('',(#79078,#79079,#79080,#79081,#79082));
#17381=EDGE_LOOP('',(#79083,#79084,#79085,#79086));
#17382=EDGE_LOOP('',(#79087,#79088,#79089,#79090));
#17383=EDGE_LOOP('',(#79091,#79092,#79093,#79094,#79095));
#17384=EDGE_LOOP('',(#79096,#79097,#79098,#79099));
#17385=EDGE_LOOP('',(#79100,#79101,#79102,#79103));
#17386=EDGE_LOOP('',(#79104,#79105,#79106,#79107));
#17387=EDGE_LOOP('',(#79108,#79109,#79110,#79111));
#17388=EDGE_LOOP('',(#79112,#79113,#79114,#79115,#79116));
#17389=EDGE_LOOP('',(#79117,#79118,#79119,#79120));
#17390=EDGE_LOOP('',(#79121,#79122,#79123,#79124));
#17391=EDGE_LOOP('',(#79125,#79126,#79127,#79128));
#17392=EDGE_LOOP('',(#79129,#79130,#79131,#79132));
#17393=EDGE_LOOP('',(#79133,#79134,#79135,#79136));
#17394=EDGE_LOOP('',(#79137,#79138,#79139,#79140));
#17395=EDGE_LOOP('',(#79141,#79142,#79143,#79144));
#17396=EDGE_LOOP('',(#79145,#79146,#79147,#79148));
#17397=EDGE_LOOP('',(#79149,#79150,#79151,#79152));
#17398=EDGE_LOOP('',(#79153,#79154,#79155,#79156));
#17399=EDGE_LOOP('',(#79157,#79158,#79159,#79160,#79161));
#17400=EDGE_LOOP('',(#79162,#79163,#79164,#79165));
#17401=EDGE_LOOP('',(#79166,#79167,#79168,#79169));
#17402=EDGE_LOOP('',(#79170,#79171,#79172,#79173));
#17403=EDGE_LOOP('',(#79174,#79175,#79176,#79177));
#17404=EDGE_LOOP('',(#79178,#79179,#79180,#79181));
#17405=EDGE_LOOP('',(#79182,#79183,#79184,#79185));
#17406=EDGE_LOOP('',(#79186,#79187,#79188,#79189));
#17407=EDGE_LOOP('',(#79190,#79191,#79192,#79193));
#17408=EDGE_LOOP('',(#79194,#79195,#79196,#79197,#79198));
#17409=EDGE_LOOP('',(#79199,#79200,#79201,#79202));
#17410=EDGE_LOOP('',(#79203,#79204,#79205,#79206));
#17411=EDGE_LOOP('',(#79207,#79208,#79209,#79210,#79211));
#17412=EDGE_LOOP('',(#79212,#79213,#79214,#79215));
#17413=EDGE_LOOP('',(#79216,#79217,#79218,#79219));
#17414=EDGE_LOOP('',(#79220,#79221,#79222,#79223));
#17415=EDGE_LOOP('',(#79224,#79225,#79226,#79227));
#17416=EDGE_LOOP('',(#79228,#79229,#79230,#79231,#79232));
#17417=EDGE_LOOP('',(#79233,#79234,#79235,#79236));
#17418=EDGE_LOOP('',(#79237,#79238,#79239,#79240));
#17419=EDGE_LOOP('',(#79241,#79242,#79243,#79244));
#17420=EDGE_LOOP('',(#79245,#79246,#79247,#79248));
#17421=EDGE_LOOP('',(#79249,#79250,#79251,#79252));
#17422=EDGE_LOOP('',(#79253,#79254,#79255,#79256));
#17423=EDGE_LOOP('',(#79257,#79258,#79259,#79260));
#17424=EDGE_LOOP('',(#79261,#79262,#79263,#79264));
#17425=EDGE_LOOP('',(#79265,#79266,#79267,#79268));
#17426=EDGE_LOOP('',(#79269,#79270,#79271,#79272));
#17427=EDGE_LOOP('',(#79273,#79274,#79275,#79276,#79277));
#17428=EDGE_LOOP('',(#79278,#79279,#79280,#79281));
#17429=EDGE_LOOP('',(#79282,#79283,#79284,#79285));
#17430=EDGE_LOOP('',(#79286,#79287,#79288,#79289));
#17431=EDGE_LOOP('',(#79290,#79291,#79292,#79293));
#17432=EDGE_LOOP('',(#79294,#79295,#79296,#79297));
#17433=EDGE_LOOP('',(#79298,#79299,#79300,#79301));
#17434=EDGE_LOOP('',(#79302,#79303,#79304,#79305));
#17435=EDGE_LOOP('',(#79306,#79307,#79308,#79309));
#17436=EDGE_LOOP('',(#79310,#79311,#79312,#79313,#79314));
#17437=EDGE_LOOP('',(#79315,#79316,#79317,#79318));
#17438=EDGE_LOOP('',(#79319,#79320,#79321,#79322));
#17439=EDGE_LOOP('',(#79323,#79324,#79325,#79326,#79327));
#17440=EDGE_LOOP('',(#79328,#79329,#79330,#79331));
#17441=EDGE_LOOP('',(#79332,#79333,#79334,#79335));
#17442=EDGE_LOOP('',(#79336,#79337,#79338,#79339));
#17443=EDGE_LOOP('',(#79340,#79341,#79342,#79343));
#17444=EDGE_LOOP('',(#79344,#79345,#79346,#79347,#79348));
#17445=EDGE_LOOP('',(#79349,#79350,#79351,#79352));
#17446=EDGE_LOOP('',(#79353,#79354,#79355,#79356));
#17447=EDGE_LOOP('',(#79357,#79358,#79359,#79360));
#17448=EDGE_LOOP('',(#79361,#79362,#79363,#79364));
#17449=EDGE_LOOP('',(#79365,#79366,#79367,#79368));
#17450=EDGE_LOOP('',(#79369,#79370,#79371,#79372));
#17451=EDGE_LOOP('',(#79373,#79374,#79375,#79376));
#17452=EDGE_LOOP('',(#79377,#79378,#79379,#79380));
#17453=EDGE_LOOP('',(#79381,#79382,#79383,#79384));
#17454=EDGE_LOOP('',(#79385,#79386,#79387,#79388));
#17455=EDGE_LOOP('',(#79389,#79390,#79391,#79392,#79393));
#17456=EDGE_LOOP('',(#79394,#79395,#79396,#79397));
#17457=EDGE_LOOP('',(#79398,#79399,#79400,#79401));
#17458=EDGE_LOOP('',(#79402,#79403,#79404,#79405));
#17459=EDGE_LOOP('',(#79406,#79407,#79408,#79409));
#17460=EDGE_LOOP('',(#79410,#79411,#79412,#79413));
#17461=EDGE_LOOP('',(#79414,#79415,#79416,#79417));
#17462=EDGE_LOOP('',(#79418,#79419,#79420,#79421));
#17463=EDGE_LOOP('',(#79422,#79423,#79424,#79425));
#17464=EDGE_LOOP('',(#79426,#79427,#79428,#79429,#79430));
#17465=EDGE_LOOP('',(#79431,#79432,#79433,#79434));
#17466=EDGE_LOOP('',(#79435,#79436,#79437,#79438));
#17467=EDGE_LOOP('',(#79439,#79440,#79441,#79442,#79443));
#17468=EDGE_LOOP('',(#79444,#79445,#79446,#79447));
#17469=EDGE_LOOP('',(#79448,#79449,#79450,#79451));
#17470=EDGE_LOOP('',(#79452,#79453,#79454,#79455));
#17471=EDGE_LOOP('',(#79456,#79457,#79458,#79459));
#17472=EDGE_LOOP('',(#79460,#79461,#79462,#79463,#79464));
#17473=EDGE_LOOP('',(#79465,#79466,#79467,#79468));
#17474=EDGE_LOOP('',(#79469,#79470,#79471,#79472));
#17475=EDGE_LOOP('',(#79473,#79474,#79475,#79476));
#17476=EDGE_LOOP('',(#79477,#79478,#79479,#79480));
#17477=EDGE_LOOP('',(#79481,#79482,#79483,#79484));
#17478=EDGE_LOOP('',(#79485,#79486,#79487,#79488));
#17479=EDGE_LOOP('',(#79489,#79490,#79491,#79492));
#17480=EDGE_LOOP('',(#79493,#79494,#79495,#79496));
#17481=EDGE_LOOP('',(#79497,#79498,#79499,#79500));
#17482=EDGE_LOOP('',(#79501,#79502,#79503,#79504));
#17483=EDGE_LOOP('',(#79505,#79506,#79507,#79508,#79509));
#17484=EDGE_LOOP('',(#79510,#79511,#79512,#79513));
#17485=EDGE_LOOP('',(#79514,#79515,#79516,#79517));
#17486=EDGE_LOOP('',(#79518,#79519,#79520,#79521));
#17487=EDGE_LOOP('',(#79522,#79523,#79524,#79525));
#17488=EDGE_LOOP('',(#79526,#79527,#79528,#79529));
#17489=EDGE_LOOP('',(#79530,#79531,#79532,#79533));
#17490=EDGE_LOOP('',(#79534,#79535,#79536,#79537));
#17491=EDGE_LOOP('',(#79538,#79539,#79540,#79541));
#17492=EDGE_LOOP('',(#79542,#79543,#79544,#79545,#79546));
#17493=EDGE_LOOP('',(#79547,#79548,#79549,#79550));
#17494=EDGE_LOOP('',(#79551,#79552,#79553,#79554));
#17495=EDGE_LOOP('',(#79555,#79556,#79557,#79558,#79559));
#17496=EDGE_LOOP('',(#79560,#79561,#79562,#79563));
#17497=EDGE_LOOP('',(#79564,#79565,#79566,#79567));
#17498=EDGE_LOOP('',(#79568,#79569,#79570,#79571));
#17499=EDGE_LOOP('',(#79572,#79573,#79574,#79575));
#17500=EDGE_LOOP('',(#79576,#79577,#79578,#79579,#79580));
#17501=EDGE_LOOP('',(#79581,#79582,#79583,#79584));
#17502=EDGE_LOOP('',(#79585,#79586,#79587,#79588));
#17503=EDGE_LOOP('',(#79589,#79590,#79591,#79592));
#17504=EDGE_LOOP('',(#79593,#79594,#79595,#79596));
#17505=EDGE_LOOP('',(#79597,#79598,#79599,#79600));
#17506=EDGE_LOOP('',(#79601,#79602,#79603,#79604));
#17507=EDGE_LOOP('',(#79605,#79606,#79607,#79608));
#17508=EDGE_LOOP('',(#79609,#79610,#79611,#79612));
#17509=EDGE_LOOP('',(#79613,#79614,#79615,#79616));
#17510=EDGE_LOOP('',(#79617,#79618,#79619,#79620));
#17511=EDGE_LOOP('',(#79621,#79622,#79623,#79624,#79625));
#17512=EDGE_LOOP('',(#79626,#79627,#79628,#79629));
#17513=EDGE_LOOP('',(#79630,#79631,#79632,#79633));
#17514=EDGE_LOOP('',(#79634,#79635,#79636,#79637));
#17515=EDGE_LOOP('',(#79638,#79639,#79640,#79641));
#17516=EDGE_LOOP('',(#79642,#79643,#79644,#79645));
#17517=EDGE_LOOP('',(#79646,#79647,#79648,#79649));
#17518=EDGE_LOOP('',(#79650,#79651,#79652,#79653));
#17519=EDGE_LOOP('',(#79654,#79655,#79656,#79657));
#17520=EDGE_LOOP('',(#79658,#79659,#79660,#79661,#79662));
#17521=EDGE_LOOP('',(#79663,#79664,#79665,#79666));
#17522=EDGE_LOOP('',(#79667,#79668,#79669,#79670));
#17523=EDGE_LOOP('',(#79671,#79672,#79673,#79674,#79675));
#17524=EDGE_LOOP('',(#79676,#79677,#79678,#79679));
#17525=EDGE_LOOP('',(#79680,#79681,#79682,#79683));
#17526=EDGE_LOOP('',(#79684,#79685,#79686,#79687));
#17527=EDGE_LOOP('',(#79688,#79689,#79690,#79691));
#17528=EDGE_LOOP('',(#79692,#79693,#79694,#79695,#79696));
#17529=EDGE_LOOP('',(#79697,#79698,#79699,#79700));
#17530=EDGE_LOOP('',(#79701,#79702,#79703,#79704));
#17531=EDGE_LOOP('',(#79705,#79706,#79707,#79708));
#17532=EDGE_LOOP('',(#79709,#79710,#79711,#79712));
#17533=EDGE_LOOP('',(#79713,#79714,#79715,#79716));
#17534=EDGE_LOOP('',(#79717,#79718,#79719,#79720));
#17535=EDGE_LOOP('',(#79721,#79722,#79723,#79724));
#17536=EDGE_LOOP('',(#79725,#79726,#79727,#79728));
#17537=EDGE_LOOP('',(#79729,#79730,#79731,#79732));
#17538=EDGE_LOOP('',(#79733,#79734,#79735,#79736));
#17539=EDGE_LOOP('',(#79737,#79738,#79739,#79740,#79741));
#17540=EDGE_LOOP('',(#79742,#79743,#79744,#79745));
#17541=EDGE_LOOP('',(#79746,#79747,#79748,#79749));
#17542=EDGE_LOOP('',(#79750,#79751,#79752,#79753));
#17543=EDGE_LOOP('',(#79754,#79755,#79756,#79757));
#17544=EDGE_LOOP('',(#79758,#79759,#79760,#79761));
#17545=EDGE_LOOP('',(#79762,#79763,#79764,#79765));
#17546=EDGE_LOOP('',(#79766,#79767,#79768,#79769));
#17547=EDGE_LOOP('',(#79770,#79771,#79772,#79773));
#17548=EDGE_LOOP('',(#79774,#79775,#79776,#79777,#79778));
#17549=EDGE_LOOP('',(#79779,#79780,#79781,#79782));
#17550=EDGE_LOOP('',(#79783,#79784,#79785,#79786));
#17551=EDGE_LOOP('',(#79787,#79788,#79789,#79790,#79791));
#17552=EDGE_LOOP('',(#79792,#79793,#79794,#79795));
#17553=EDGE_LOOP('',(#79796,#79797,#79798,#79799));
#17554=EDGE_LOOP('',(#79800,#79801,#79802,#79803));
#17555=EDGE_LOOP('',(#79804,#79805,#79806,#79807));
#17556=EDGE_LOOP('',(#79808,#79809,#79810,#79811,#79812));
#17557=EDGE_LOOP('',(#79813,#79814,#79815,#79816));
#17558=EDGE_LOOP('',(#79817,#79818,#79819,#79820));
#17559=EDGE_LOOP('',(#79821,#79822,#79823,#79824));
#17560=EDGE_LOOP('',(#79825,#79826,#79827,#79828));
#17561=EDGE_LOOP('',(#79829,#79830,#79831,#79832));
#17562=EDGE_LOOP('',(#79833,#79834,#79835,#79836));
#17563=EDGE_LOOP('',(#79837,#79838,#79839,#79840));
#17564=EDGE_LOOP('',(#79841,#79842,#79843,#79844));
#17565=EDGE_LOOP('',(#79845,#79846,#79847,#79848));
#17566=EDGE_LOOP('',(#79849,#79850,#79851,#79852));
#17567=EDGE_LOOP('',(#79853,#79854,#79855,#79856,#79857));
#17568=EDGE_LOOP('',(#79858,#79859,#79860,#79861));
#17569=EDGE_LOOP('',(#79862,#79863,#79864,#79865));
#17570=EDGE_LOOP('',(#79866,#79867,#79868,#79869));
#17571=EDGE_LOOP('',(#79870,#79871,#79872,#79873));
#17572=EDGE_LOOP('',(#79874,#79875,#79876,#79877));
#17573=EDGE_LOOP('',(#79878,#79879,#79880,#79881));
#17574=EDGE_LOOP('',(#79882,#79883,#79884,#79885));
#17575=EDGE_LOOP('',(#79886,#79887,#79888,#79889));
#17576=EDGE_LOOP('',(#79890,#79891,#79892,#79893,#79894));
#17577=EDGE_LOOP('',(#79895,#79896,#79897,#79898));
#17578=EDGE_LOOP('',(#79899,#79900,#79901,#79902));
#17579=EDGE_LOOP('',(#79903,#79904,#79905,#79906,#79907));
#17580=EDGE_LOOP('',(#79908,#79909,#79910,#79911));
#17581=EDGE_LOOP('',(#79912,#79913,#79914,#79915));
#17582=EDGE_LOOP('',(#79916,#79917,#79918,#79919));
#17583=EDGE_LOOP('',(#79920,#79921,#79922,#79923));
#17584=EDGE_LOOP('',(#79924,#79925,#79926,#79927,#79928));
#17585=EDGE_LOOP('',(#79929,#79930,#79931,#79932));
#17586=EDGE_LOOP('',(#79933,#79934,#79935,#79936));
#17587=EDGE_LOOP('',(#79937,#79938,#79939,#79940));
#17588=EDGE_LOOP('',(#79941,#79942,#79943,#79944));
#17589=EDGE_LOOP('',(#79945,#79946,#79947,#79948));
#17590=EDGE_LOOP('',(#79949,#79950,#79951,#79952));
#17591=EDGE_LOOP('',(#79953,#79954,#79955,#79956));
#17592=EDGE_LOOP('',(#79957,#79958,#79959,#79960));
#17593=EDGE_LOOP('',(#79961,#79962,#79963,#79964));
#17594=EDGE_LOOP('',(#79965,#79966,#79967,#79968));
#17595=EDGE_LOOP('',(#79969,#79970,#79971,#79972,#79973));
#17596=EDGE_LOOP('',(#79974,#79975,#79976,#79977));
#17597=EDGE_LOOP('',(#79978,#79979,#79980,#79981));
#17598=EDGE_LOOP('',(#79982,#79983,#79984,#79985));
#17599=EDGE_LOOP('',(#79986,#79987,#79988,#79989));
#17600=EDGE_LOOP('',(#79990,#79991,#79992,#79993));
#17601=EDGE_LOOP('',(#79994,#79995,#79996,#79997));
#17602=EDGE_LOOP('',(#79998,#79999,#80000,#80001));
#17603=EDGE_LOOP('',(#80002,#80003,#80004,#80005));
#17604=EDGE_LOOP('',(#80006,#80007,#80008,#80009,#80010));
#17605=EDGE_LOOP('',(#80011,#80012,#80013,#80014));
#17606=EDGE_LOOP('',(#80015,#80016,#80017,#80018));
#17607=EDGE_LOOP('',(#80019,#80020,#80021,#80022,#80023));
#17608=EDGE_LOOP('',(#80024,#80025,#80026,#80027));
#17609=EDGE_LOOP('',(#80028,#80029,#80030,#80031));
#17610=EDGE_LOOP('',(#80032,#80033,#80034,#80035));
#17611=EDGE_LOOP('',(#80036,#80037,#80038,#80039));
#17612=EDGE_LOOP('',(#80040,#80041,#80042,#80043,#80044));
#17613=EDGE_LOOP('',(#80045,#80046,#80047,#80048));
#17614=EDGE_LOOP('',(#80049,#80050,#80051,#80052));
#17615=EDGE_LOOP('',(#80053,#80054,#80055,#80056));
#17616=EDGE_LOOP('',(#80057,#80058,#80059,#80060));
#17617=EDGE_LOOP('',(#80061,#80062,#80063,#80064));
#17618=EDGE_LOOP('',(#80065,#80066,#80067,#80068));
#17619=EDGE_LOOP('',(#80069,#80070,#80071,#80072));
#17620=EDGE_LOOP('',(#80073,#80074,#80075,#80076));
#17621=EDGE_LOOP('',(#80077,#80078,#80079,#80080));
#17622=EDGE_LOOP('',(#80081,#80082,#80083,#80084));
#17623=EDGE_LOOP('',(#80085,#80086,#80087,#80088,#80089));
#17624=EDGE_LOOP('',(#80090,#80091,#80092,#80093));
#17625=EDGE_LOOP('',(#80094,#80095,#80096,#80097));
#17626=EDGE_LOOP('',(#80098,#80099,#80100,#80101));
#17627=EDGE_LOOP('',(#80102,#80103,#80104,#80105));
#17628=EDGE_LOOP('',(#80106,#80107,#80108,#80109));
#17629=EDGE_LOOP('',(#80110,#80111,#80112,#80113));
#17630=EDGE_LOOP('',(#80114,#80115,#80116,#80117));
#17631=EDGE_LOOP('',(#80118,#80119,#80120,#80121));
#17632=EDGE_LOOP('',(#80122,#80123,#80124,#80125,#80126));
#17633=EDGE_LOOP('',(#80127,#80128,#80129,#80130));
#17634=EDGE_LOOP('',(#80131,#80132,#80133,#80134));
#17635=EDGE_LOOP('',(#80135,#80136,#80137,#80138,#80139));
#17636=EDGE_LOOP('',(#80140,#80141,#80142,#80143));
#17637=EDGE_LOOP('',(#80144,#80145,#80146,#80147));
#17638=EDGE_LOOP('',(#80148,#80149,#80150,#80151));
#17639=EDGE_LOOP('',(#80152,#80153,#80154,#80155));
#17640=EDGE_LOOP('',(#80156,#80157,#80158,#80159,#80160));
#17641=EDGE_LOOP('',(#80161,#80162,#80163,#80164));
#17642=EDGE_LOOP('',(#80165,#80166,#80167,#80168));
#17643=EDGE_LOOP('',(#80169,#80170,#80171,#80172));
#17644=EDGE_LOOP('',(#80173,#80174,#80175,#80176));
#17645=EDGE_LOOP('',(#80177,#80178,#80179,#80180));
#17646=EDGE_LOOP('',(#80181,#80182,#80183,#80184));
#17647=EDGE_LOOP('',(#80185,#80186,#80187,#80188));
#17648=EDGE_LOOP('',(#80189,#80190,#80191,#80192));
#17649=EDGE_LOOP('',(#80193,#80194,#80195,#80196));
#17650=EDGE_LOOP('',(#80197,#80198,#80199,#80200));
#17651=EDGE_LOOP('',(#80201,#80202,#80203,#80204,#80205));
#17652=EDGE_LOOP('',(#80206,#80207,#80208,#80209));
#17653=EDGE_LOOP('',(#80210,#80211,#80212,#80213));
#17654=EDGE_LOOP('',(#80214,#80215,#80216,#80217));
#17655=EDGE_LOOP('',(#80218,#80219,#80220,#80221));
#17656=EDGE_LOOP('',(#80222,#80223,#80224,#80225));
#17657=EDGE_LOOP('',(#80226,#80227,#80228,#80229));
#17658=EDGE_LOOP('',(#80230,#80231,#80232,#80233));
#17659=EDGE_LOOP('',(#80234,#80235,#80236,#80237));
#17660=EDGE_LOOP('',(#80238,#80239,#80240,#80241,#80242));
#17661=EDGE_LOOP('',(#80243,#80244,#80245,#80246));
#17662=EDGE_LOOP('',(#80247,#80248,#80249,#80250));
#17663=EDGE_LOOP('',(#80251,#80252,#80253,#80254,#80255));
#17664=EDGE_LOOP('',(#80256,#80257,#80258,#80259));
#17665=EDGE_LOOP('',(#80260,#80261,#80262,#80263));
#17666=EDGE_LOOP('',(#80264,#80265,#80266,#80267));
#17667=EDGE_LOOP('',(#80268,#80269,#80270,#80271));
#17668=EDGE_LOOP('',(#80272,#80273,#80274,#80275,#80276));
#17669=EDGE_LOOP('',(#80277,#80278,#80279,#80280));
#17670=EDGE_LOOP('',(#80281,#80282,#80283,#80284));
#17671=EDGE_LOOP('',(#80285,#80286,#80287,#80288));
#17672=EDGE_LOOP('',(#80289,#80290,#80291,#80292));
#17673=EDGE_LOOP('',(#80293,#80294,#80295,#80296));
#17674=EDGE_LOOP('',(#80297,#80298,#80299,#80300));
#17675=EDGE_LOOP('',(#80301,#80302,#80303,#80304));
#17676=EDGE_LOOP('',(#80305,#80306,#80307,#80308));
#17677=EDGE_LOOP('',(#80309,#80310,#80311,#80312));
#17678=EDGE_LOOP('',(#80313,#80314,#80315,#80316));
#17679=EDGE_LOOP('',(#80317,#80318,#80319,#80320,#80321));
#17680=EDGE_LOOP('',(#80322,#80323,#80324,#80325));
#17681=EDGE_LOOP('',(#80326,#80327,#80328,#80329));
#17682=EDGE_LOOP('',(#80330,#80331,#80332,#80333));
#17683=EDGE_LOOP('',(#80334,#80335,#80336,#80337));
#17684=EDGE_LOOP('',(#80338,#80339,#80340,#80341));
#17685=EDGE_LOOP('',(#80342,#80343,#80344,#80345));
#17686=EDGE_LOOP('',(#80346,#80347,#80348,#80349));
#17687=EDGE_LOOP('',(#80350,#80351,#80352,#80353));
#17688=EDGE_LOOP('',(#80354,#80355,#80356,#80357,#80358));
#17689=EDGE_LOOP('',(#80359,#80360,#80361,#80362));
#17690=EDGE_LOOP('',(#80363,#80364,#80365,#80366));
#17691=EDGE_LOOP('',(#80367,#80368,#80369,#80370,#80371));
#17692=EDGE_LOOP('',(#80372,#80373,#80374,#80375));
#17693=EDGE_LOOP('',(#80376,#80377,#80378,#80379));
#17694=EDGE_LOOP('',(#80380,#80381,#80382,#80383));
#17695=EDGE_LOOP('',(#80384,#80385,#80386,#80387));
#17696=EDGE_LOOP('',(#80388,#80389,#80390,#80391,#80392));
#17697=EDGE_LOOP('',(#80393,#80394,#80395,#80396));
#17698=EDGE_LOOP('',(#80397,#80398,#80399,#80400));
#17699=EDGE_LOOP('',(#80401,#80402,#80403,#80404));
#17700=EDGE_LOOP('',(#80405,#80406,#80407,#80408));
#17701=EDGE_LOOP('',(#80409,#80410,#80411,#80412));
#17702=EDGE_LOOP('',(#80413,#80414,#80415,#80416));
#17703=EDGE_LOOP('',(#80417,#80418,#80419,#80420));
#17704=EDGE_LOOP('',(#80421,#80422,#80423,#80424));
#17705=EDGE_LOOP('',(#80425,#80426,#80427,#80428));
#17706=EDGE_LOOP('',(#80429,#80430,#80431,#80432));
#17707=EDGE_LOOP('',(#80433,#80434,#80435,#80436,#80437));
#17708=EDGE_LOOP('',(#80438,#80439,#80440,#80441));
#17709=EDGE_LOOP('',(#80442,#80443,#80444,#80445));
#17710=EDGE_LOOP('',(#80446,#80447,#80448,#80449));
#17711=EDGE_LOOP('',(#80450,#80451,#80452,#80453));
#17712=EDGE_LOOP('',(#80454,#80455,#80456,#80457));
#17713=EDGE_LOOP('',(#80458,#80459,#80460,#80461));
#17714=EDGE_LOOP('',(#80462,#80463,#80464,#80465));
#17715=EDGE_LOOP('',(#80466,#80467,#80468,#80469));
#17716=EDGE_LOOP('',(#80470,#80471,#80472,#80473,#80474));
#17717=EDGE_LOOP('',(#80475,#80476,#80477,#80478));
#17718=EDGE_LOOP('',(#80479,#80480,#80481,#80482));
#17719=EDGE_LOOP('',(#80483,#80484,#80485,#80486,#80487));
#17720=EDGE_LOOP('',(#80488,#80489,#80490,#80491));
#17721=EDGE_LOOP('',(#80492,#80493,#80494,#80495));
#17722=EDGE_LOOP('',(#80496,#80497,#80498,#80499));
#17723=EDGE_LOOP('',(#80500,#80501,#80502,#80503));
#17724=EDGE_LOOP('',(#80504,#80505,#80506,#80507,#80508));
#17725=EDGE_LOOP('',(#80509,#80510,#80511,#80512));
#17726=EDGE_LOOP('',(#80513,#80514,#80515,#80516));
#17727=EDGE_LOOP('',(#80517,#80518,#80519,#80520));
#17728=EDGE_LOOP('',(#80521,#80522,#80523,#80524));
#17729=EDGE_LOOP('',(#80525,#80526,#80527,#80528));
#17730=EDGE_LOOP('',(#80529,#80530,#80531,#80532));
#17731=EDGE_LOOP('',(#80533,#80534,#80535,#80536));
#17732=EDGE_LOOP('',(#80537,#80538,#80539,#80540));
#17733=EDGE_LOOP('',(#80541,#80542,#80543,#80544));
#17734=EDGE_LOOP('',(#80545,#80546,#80547,#80548));
#17735=EDGE_LOOP('',(#80549,#80550,#80551,#80552,#80553));
#17736=EDGE_LOOP('',(#80554,#80555,#80556,#80557));
#17737=EDGE_LOOP('',(#80558,#80559,#80560,#80561));
#17738=EDGE_LOOP('',(#80562,#80563,#80564,#80565));
#17739=EDGE_LOOP('',(#80566,#80567,#80568,#80569));
#17740=EDGE_LOOP('',(#80570,#80571,#80572,#80573));
#17741=EDGE_LOOP('',(#80574,#80575,#80576,#80577));
#17742=EDGE_LOOP('',(#80578,#80579,#80580,#80581));
#17743=EDGE_LOOP('',(#80582,#80583,#80584,#80585));
#17744=EDGE_LOOP('',(#80586,#80587,#80588,#80589,#80590));
#17745=EDGE_LOOP('',(#80591,#80592,#80593,#80594));
#17746=EDGE_LOOP('',(#80595,#80596,#80597,#80598));
#17747=EDGE_LOOP('',(#80599,#80600,#80601,#80602,#80603));
#17748=EDGE_LOOP('',(#80604,#80605,#80606,#80607));
#17749=EDGE_LOOP('',(#80608,#80609,#80610,#80611));
#17750=EDGE_LOOP('',(#80612,#80613,#80614,#80615));
#17751=EDGE_LOOP('',(#80616,#80617,#80618,#80619));
#17752=EDGE_LOOP('',(#80620,#80621,#80622,#80623,#80624));
#17753=EDGE_LOOP('',(#80625,#80626,#80627,#80628));
#17754=EDGE_LOOP('',(#80629,#80630,#80631,#80632));
#17755=EDGE_LOOP('',(#80633,#80634,#80635,#80636));
#17756=EDGE_LOOP('',(#80637,#80638,#80639,#80640));
#17757=EDGE_LOOP('',(#80641,#80642,#80643,#80644));
#17758=EDGE_LOOP('',(#80645,#80646,#80647,#80648));
#17759=EDGE_LOOP('',(#80649,#80650,#80651,#80652));
#17760=EDGE_LOOP('',(#80653,#80654,#80655,#80656));
#17761=EDGE_LOOP('',(#80657,#80658,#80659,#80660));
#17762=EDGE_LOOP('',(#80661,#80662,#80663,#80664));
#17763=EDGE_LOOP('',(#80665,#80666,#80667,#80668,#80669));
#17764=EDGE_LOOP('',(#80670,#80671,#80672,#80673));
#17765=EDGE_LOOP('',(#80674,#80675,#80676,#80677));
#17766=EDGE_LOOP('',(#80678,#80679,#80680,#80681));
#17767=EDGE_LOOP('',(#80682,#80683,#80684,#80685));
#17768=EDGE_LOOP('',(#80686,#80687,#80688,#80689));
#17769=EDGE_LOOP('',(#80690,#80691,#80692,#80693));
#17770=EDGE_LOOP('',(#80694,#80695,#80696,#80697));
#17771=EDGE_LOOP('',(#80698,#80699,#80700,#80701));
#17772=EDGE_LOOP('',(#80702,#80703,#80704,#80705,#80706));
#17773=EDGE_LOOP('',(#80707,#80708,#80709,#80710));
#17774=EDGE_LOOP('',(#80711,#80712,#80713,#80714));
#17775=EDGE_LOOP('',(#80715,#80716,#80717,#80718,#80719));
#17776=EDGE_LOOP('',(#80720,#80721,#80722,#80723));
#17777=EDGE_LOOP('',(#80724,#80725,#80726,#80727));
#17778=EDGE_LOOP('',(#80728,#80729,#80730,#80731));
#17779=EDGE_LOOP('',(#80732,#80733,#80734,#80735));
#17780=EDGE_LOOP('',(#80736,#80737,#80738,#80739,#80740));
#17781=EDGE_LOOP('',(#80741,#80742,#80743,#80744));
#17782=EDGE_LOOP('',(#80745,#80746,#80747,#80748));
#17783=EDGE_LOOP('',(#80749,#80750,#80751,#80752));
#17784=EDGE_LOOP('',(#80753,#80754,#80755,#80756));
#17785=EDGE_LOOP('',(#80757,#80758,#80759,#80760));
#17786=EDGE_LOOP('',(#80761,#80762,#80763,#80764));
#17787=EDGE_LOOP('',(#80765,#80766,#80767,#80768));
#17788=EDGE_LOOP('',(#80769,#80770,#80771,#80772));
#17789=EDGE_LOOP('',(#80773,#80774,#80775,#80776));
#17790=EDGE_LOOP('',(#80777,#80778,#80779,#80780));
#17791=EDGE_LOOP('',(#80781,#80782,#80783,#80784,#80785));
#17792=EDGE_LOOP('',(#80786,#80787,#80788,#80789));
#17793=EDGE_LOOP('',(#80790,#80791,#80792,#80793));
#17794=EDGE_LOOP('',(#80794,#80795,#80796,#80797));
#17795=EDGE_LOOP('',(#80798,#80799,#80800,#80801));
#17796=EDGE_LOOP('',(#80802,#80803,#80804,#80805));
#17797=EDGE_LOOP('',(#80806,#80807,#80808,#80809));
#17798=EDGE_LOOP('',(#80810,#80811,#80812,#80813));
#17799=EDGE_LOOP('',(#80814,#80815,#80816,#80817));
#17800=EDGE_LOOP('',(#80818,#80819,#80820,#80821,#80822));
#17801=EDGE_LOOP('',(#80823,#80824,#80825,#80826));
#17802=EDGE_LOOP('',(#80827,#80828,#80829,#80830));
#17803=EDGE_LOOP('',(#80831,#80832,#80833,#80834,#80835));
#17804=EDGE_LOOP('',(#80836,#80837,#80838,#80839));
#17805=EDGE_LOOP('',(#80840,#80841,#80842,#80843));
#17806=EDGE_LOOP('',(#80844,#80845,#80846,#80847));
#17807=EDGE_LOOP('',(#80848,#80849,#80850,#80851));
#17808=EDGE_LOOP('',(#80852,#80853,#80854,#80855,#80856));
#17809=EDGE_LOOP('',(#80857,#80858,#80859,#80860));
#17810=EDGE_LOOP('',(#80861,#80862,#80863,#80864));
#17811=EDGE_LOOP('',(#80865,#80866,#80867,#80868));
#17812=EDGE_LOOP('',(#80869,#80870,#80871,#80872));
#17813=EDGE_LOOP('',(#80873,#80874,#80875,#80876));
#17814=EDGE_LOOP('',(#80877,#80878,#80879,#80880));
#17815=EDGE_LOOP('',(#80881,#80882,#80883,#80884));
#17816=EDGE_LOOP('',(#80885,#80886,#80887,#80888));
#17817=EDGE_LOOP('',(#80889,#80890,#80891,#80892));
#17818=EDGE_LOOP('',(#80893,#80894,#80895,#80896));
#17819=EDGE_LOOP('',(#80897,#80898,#80899,#80900,#80901));
#17820=EDGE_LOOP('',(#80902,#80903,#80904,#80905));
#17821=EDGE_LOOP('',(#80906,#80907,#80908,#80909));
#17822=EDGE_LOOP('',(#80910,#80911,#80912,#80913));
#17823=EDGE_LOOP('',(#80914,#80915,#80916,#80917));
#17824=EDGE_LOOP('',(#80918,#80919,#80920,#80921));
#17825=EDGE_LOOP('',(#80922,#80923,#80924,#80925));
#17826=EDGE_LOOP('',(#80926,#80927,#80928,#80929));
#17827=EDGE_LOOP('',(#80930,#80931,#80932,#80933));
#17828=EDGE_LOOP('',(#80934,#80935,#80936,#80937,#80938));
#17829=EDGE_LOOP('',(#80939,#80940,#80941,#80942));
#17830=EDGE_LOOP('',(#80943,#80944,#80945,#80946));
#17831=EDGE_LOOP('',(#80947,#80948,#80949,#80950,#80951));
#17832=EDGE_LOOP('',(#80952,#80953,#80954,#80955));
#17833=EDGE_LOOP('',(#80956,#80957,#80958,#80959));
#17834=EDGE_LOOP('',(#80960,#80961,#80962,#80963));
#17835=EDGE_LOOP('',(#80964,#80965,#80966,#80967));
#17836=EDGE_LOOP('',(#80968,#80969,#80970,#80971,#80972));
#17837=EDGE_LOOP('',(#80973,#80974,#80975,#80976));
#17838=EDGE_LOOP('',(#80977,#80978,#80979,#80980));
#17839=EDGE_LOOP('',(#80981,#80982,#80983,#80984));
#17840=EDGE_LOOP('',(#80985,#80986,#80987,#80988));
#17841=EDGE_LOOP('',(#80989,#80990,#80991,#80992));
#17842=EDGE_LOOP('',(#80993,#80994,#80995,#80996));
#17843=EDGE_LOOP('',(#80997,#80998,#80999,#81000));
#17844=EDGE_LOOP('',(#81001,#81002,#81003,#81004));
#17845=EDGE_LOOP('',(#81005,#81006,#81007,#81008));
#17846=EDGE_LOOP('',(#81009,#81010,#81011,#81012));
#17847=EDGE_LOOP('',(#81013,#81014,#81015,#81016,#81017));
#17848=EDGE_LOOP('',(#81018,#81019,#81020,#81021));
#17849=EDGE_LOOP('',(#81022,#81023,#81024,#81025));
#17850=EDGE_LOOP('',(#81026,#81027,#81028,#81029));
#17851=EDGE_LOOP('',(#81030,#81031,#81032,#81033));
#17852=EDGE_LOOP('',(#81034,#81035,#81036,#81037));
#17853=EDGE_LOOP('',(#81038,#81039,#81040,#81041));
#17854=EDGE_LOOP('',(#81042,#81043,#81044,#81045));
#17855=EDGE_LOOP('',(#81046,#81047,#81048,#81049));
#17856=EDGE_LOOP('',(#81050,#81051,#81052,#81053,#81054));
#17857=EDGE_LOOP('',(#81055,#81056,#81057,#81058));
#17858=EDGE_LOOP('',(#81059,#81060,#81061,#81062));
#17859=EDGE_LOOP('',(#81063,#81064,#81065,#81066,#81067));
#17860=EDGE_LOOP('',(#81068,#81069,#81070,#81071));
#17861=EDGE_LOOP('',(#81072,#81073,#81074,#81075));
#17862=EDGE_LOOP('',(#81076,#81077,#81078,#81079));
#17863=EDGE_LOOP('',(#81080,#81081,#81082,#81083));
#17864=EDGE_LOOP('',(#81084,#81085,#81086,#81087,#81088));
#17865=EDGE_LOOP('',(#81089,#81090,#81091,#81092));
#17866=EDGE_LOOP('',(#81093,#81094,#81095,#81096));
#17867=EDGE_LOOP('',(#81097,#81098,#81099,#81100));
#17868=EDGE_LOOP('',(#81101,#81102,#81103,#81104));
#17869=EDGE_LOOP('',(#81105,#81106,#81107,#81108));
#17870=EDGE_LOOP('',(#81109,#81110,#81111,#81112));
#17871=EDGE_LOOP('',(#81113,#81114,#81115,#81116));
#17872=EDGE_LOOP('',(#81117,#81118,#81119,#81120));
#17873=EDGE_LOOP('',(#81121,#81122,#81123,#81124));
#17874=EDGE_LOOP('',(#81125,#81126,#81127,#81128));
#17875=EDGE_LOOP('',(#81129,#81130,#81131,#81132,#81133));
#17876=EDGE_LOOP('',(#81134,#81135,#81136,#81137));
#17877=EDGE_LOOP('',(#81138,#81139,#81140,#81141));
#17878=EDGE_LOOP('',(#81142,#81143,#81144,#81145));
#17879=EDGE_LOOP('',(#81146,#81147,#81148,#81149));
#17880=EDGE_LOOP('',(#81150,#81151,#81152,#81153));
#17881=EDGE_LOOP('',(#81154,#81155,#81156,#81157));
#17882=EDGE_LOOP('',(#81158,#81159,#81160,#81161));
#17883=EDGE_LOOP('',(#81162,#81163,#81164,#81165));
#17884=EDGE_LOOP('',(#81166,#81167,#81168,#81169,#81170));
#17885=EDGE_LOOP('',(#81171,#81172,#81173,#81174));
#17886=EDGE_LOOP('',(#81175,#81176,#81177,#81178));
#17887=EDGE_LOOP('',(#81179,#81180,#81181,#81182,#81183));
#17888=EDGE_LOOP('',(#81184,#81185,#81186,#81187));
#17889=EDGE_LOOP('',(#81188,#81189,#81190,#81191));
#17890=EDGE_LOOP('',(#81192,#81193,#81194,#81195));
#17891=EDGE_LOOP('',(#81196,#81197,#81198,#81199));
#17892=EDGE_LOOP('',(#81200,#81201,#81202,#81203,#81204));
#17893=EDGE_LOOP('',(#81205,#81206,#81207,#81208));
#17894=EDGE_LOOP('',(#81209,#81210,#81211,#81212));
#17895=EDGE_LOOP('',(#81213,#81214,#81215,#81216));
#17896=EDGE_LOOP('',(#81217,#81218,#81219,#81220));
#17897=EDGE_LOOP('',(#81221,#81222,#81223,#81224));
#17898=EDGE_LOOP('',(#81225,#81226,#81227,#81228));
#17899=EDGE_LOOP('',(#81229,#81230,#81231,#81232));
#17900=EDGE_LOOP('',(#81233,#81234,#81235,#81236));
#17901=EDGE_LOOP('',(#81237,#81238,#81239,#81240));
#17902=EDGE_LOOP('',(#81241,#81242,#81243,#81244));
#17903=EDGE_LOOP('',(#81245,#81246,#81247,#81248,#81249));
#17904=EDGE_LOOP('',(#81250,#81251,#81252,#81253));
#17905=EDGE_LOOP('',(#81254,#81255,#81256,#81257));
#17906=EDGE_LOOP('',(#81258,#81259,#81260,#81261));
#17907=EDGE_LOOP('',(#81262,#81263,#81264,#81265));
#17908=EDGE_LOOP('',(#81266,#81267,#81268,#81269));
#17909=EDGE_LOOP('',(#81270,#81271,#81272,#81273));
#17910=EDGE_LOOP('',(#81274,#81275,#81276,#81277));
#17911=EDGE_LOOP('',(#81278,#81279,#81280,#81281));
#17912=EDGE_LOOP('',(#81282,#81283,#81284,#81285,#81286));
#17913=EDGE_LOOP('',(#81287,#81288,#81289,#81290));
#17914=EDGE_LOOP('',(#81291,#81292,#81293,#81294));
#17915=EDGE_LOOP('',(#81295,#81296,#81297,#81298,#81299));
#17916=EDGE_LOOP('',(#81300,#81301,#81302,#81303));
#17917=EDGE_LOOP('',(#81304,#81305,#81306,#81307));
#17918=EDGE_LOOP('',(#81308,#81309,#81310,#81311));
#17919=EDGE_LOOP('',(#81312,#81313,#81314,#81315));
#17920=EDGE_LOOP('',(#81316,#81317,#81318,#81319,#81320));
#17921=EDGE_LOOP('',(#81321,#81322,#81323,#81324));
#17922=EDGE_LOOP('',(#81325,#81326,#81327,#81328));
#17923=EDGE_LOOP('',(#81329,#81330,#81331,#81332));
#17924=EDGE_LOOP('',(#81333,#81334,#81335,#81336));
#17925=EDGE_LOOP('',(#81337,#81338,#81339,#81340));
#17926=EDGE_LOOP('',(#81341,#81342,#81343,#81344));
#17927=EDGE_LOOP('',(#81345,#81346,#81347,#81348));
#17928=EDGE_LOOP('',(#81349,#81350,#81351,#81352));
#17929=EDGE_LOOP('',(#81353,#81354,#81355,#81356));
#17930=EDGE_LOOP('',(#81357,#81358,#81359,#81360));
#17931=EDGE_LOOP('',(#81361,#81362,#81363,#81364,#81365));
#17932=EDGE_LOOP('',(#81366,#81367,#81368,#81369));
#17933=EDGE_LOOP('',(#81370,#81371,#81372,#81373));
#17934=EDGE_LOOP('',(#81374,#81375,#81376,#81377));
#17935=EDGE_LOOP('',(#81378,#81379,#81380,#81381));
#17936=EDGE_LOOP('',(#81382,#81383,#81384,#81385));
#17937=EDGE_LOOP('',(#81386,#81387,#81388,#81389));
#17938=EDGE_LOOP('',(#81390,#81391,#81392,#81393));
#17939=EDGE_LOOP('',(#81394,#81395,#81396,#81397));
#17940=EDGE_LOOP('',(#81398,#81399,#81400,#81401,#81402));
#17941=EDGE_LOOP('',(#81403,#81404,#81405,#81406));
#17942=EDGE_LOOP('',(#81407,#81408,#81409,#81410));
#17943=EDGE_LOOP('',(#81411,#81412,#81413,#81414,#81415));
#17944=EDGE_LOOP('',(#81416,#81417,#81418,#81419));
#17945=EDGE_LOOP('',(#81420,#81421,#81422,#81423));
#17946=EDGE_LOOP('',(#81424,#81425,#81426,#81427));
#17947=EDGE_LOOP('',(#81428,#81429,#81430,#81431));
#17948=EDGE_LOOP('',(#81432,#81433,#81434,#81435,#81436));
#17949=EDGE_LOOP('',(#81437,#81438,#81439,#81440));
#17950=EDGE_LOOP('',(#81441,#81442,#81443,#81444));
#17951=EDGE_LOOP('',(#81445,#81446,#81447,#81448));
#17952=EDGE_LOOP('',(#81449,#81450,#81451,#81452));
#17953=EDGE_LOOP('',(#81453,#81454,#81455,#81456));
#17954=EDGE_LOOP('',(#81457,#81458,#81459,#81460));
#17955=EDGE_LOOP('',(#81461,#81462,#81463,#81464));
#17956=EDGE_LOOP('',(#81465,#81466,#81467,#81468));
#17957=EDGE_LOOP('',(#81469,#81470,#81471,#81472));
#17958=EDGE_LOOP('',(#81473,#81474,#81475,#81476));
#17959=EDGE_LOOP('',(#81477,#81478,#81479,#81480,#81481));
#17960=EDGE_LOOP('',(#81482,#81483,#81484,#81485));
#17961=EDGE_LOOP('',(#81486,#81487,#81488,#81489));
#17962=EDGE_LOOP('',(#81490,#81491,#81492,#81493));
#17963=EDGE_LOOP('',(#81494,#81495,#81496,#81497));
#17964=EDGE_LOOP('',(#81498,#81499,#81500,#81501));
#17965=EDGE_LOOP('',(#81502,#81503,#81504,#81505));
#17966=EDGE_LOOP('',(#81506,#81507,#81508,#81509));
#17967=EDGE_LOOP('',(#81510,#81511,#81512,#81513));
#17968=EDGE_LOOP('',(#81514,#81515,#81516,#81517,#81518));
#17969=EDGE_LOOP('',(#81519,#81520,#81521,#81522));
#17970=EDGE_LOOP('',(#81523,#81524,#81525,#81526));
#17971=EDGE_LOOP('',(#81527,#81528,#81529,#81530,#81531));
#17972=EDGE_LOOP('',(#81532,#81533,#81534,#81535));
#17973=EDGE_LOOP('',(#81536,#81537,#81538,#81539));
#17974=EDGE_LOOP('',(#81540,#81541,#81542,#81543));
#17975=EDGE_LOOP('',(#81544,#81545,#81546,#81547));
#17976=EDGE_LOOP('',(#81548,#81549,#81550,#81551,#81552));
#17977=EDGE_LOOP('',(#81553,#81554,#81555,#81556));
#17978=EDGE_LOOP('',(#81557,#81558,#81559,#81560));
#17979=EDGE_LOOP('',(#81561,#81562,#81563,#81564));
#17980=EDGE_LOOP('',(#81565,#81566,#81567,#81568));
#17981=EDGE_LOOP('',(#81569,#81570,#81571,#81572));
#17982=EDGE_LOOP('',(#81573,#81574,#81575,#81576));
#17983=EDGE_LOOP('',(#81577,#81578,#81579,#81580));
#17984=EDGE_LOOP('',(#81581,#81582,#81583,#81584));
#17985=EDGE_LOOP('',(#81585,#81586,#81587,#81588));
#17986=EDGE_LOOP('',(#81589,#81590,#81591,#81592));
#17987=EDGE_LOOP('',(#81593,#81594,#81595,#81596,#81597));
#17988=EDGE_LOOP('',(#81598,#81599,#81600,#81601));
#17989=EDGE_LOOP('',(#81602,#81603,#81604,#81605));
#17990=EDGE_LOOP('',(#81606,#81607,#81608,#81609));
#17991=EDGE_LOOP('',(#81610,#81611,#81612,#81613));
#17992=EDGE_LOOP('',(#81614,#81615,#81616,#81617));
#17993=EDGE_LOOP('',(#81618,#81619,#81620,#81621));
#17994=EDGE_LOOP('',(#81622,#81623,#81624,#81625));
#17995=EDGE_LOOP('',(#81626,#81627,#81628,#81629));
#17996=EDGE_LOOP('',(#81630,#81631,#81632,#81633,#81634));
#17997=EDGE_LOOP('',(#81635,#81636,#81637,#81638));
#17998=EDGE_LOOP('',(#81639,#81640,#81641,#81642));
#17999=EDGE_LOOP('',(#81643,#81644,#81645,#81646,#81647));
#18000=EDGE_LOOP('',(#81648,#81649,#81650,#81651));
#18001=EDGE_LOOP('',(#81652,#81653,#81654,#81655));
#18002=EDGE_LOOP('',(#81656,#81657,#81658,#81659));
#18003=EDGE_LOOP('',(#81660,#81661,#81662,#81663));
#18004=EDGE_LOOP('',(#81664,#81665,#81666,#81667,#81668));
#18005=EDGE_LOOP('',(#81669,#81670,#81671,#81672));
#18006=EDGE_LOOP('',(#81673,#81674,#81675,#81676));
#18007=EDGE_LOOP('',(#81677,#81678,#81679,#81680));
#18008=EDGE_LOOP('',(#81681,#81682,#81683,#81684));
#18009=EDGE_LOOP('',(#81685,#81686,#81687,#81688));
#18010=EDGE_LOOP('',(#81689,#81690,#81691,#81692));
#18011=EDGE_LOOP('',(#81693,#81694,#81695,#81696));
#18012=EDGE_LOOP('',(#81697,#81698,#81699,#81700));
#18013=EDGE_LOOP('',(#81701,#81702,#81703,#81704));
#18014=EDGE_LOOP('',(#81705,#81706,#81707,#81708));
#18015=EDGE_LOOP('',(#81709,#81710,#81711,#81712,#81713));
#18016=EDGE_LOOP('',(#81714,#81715,#81716,#81717));
#18017=EDGE_LOOP('',(#81718,#81719,#81720,#81721));
#18018=EDGE_LOOP('',(#81722,#81723,#81724,#81725));
#18019=EDGE_LOOP('',(#81726,#81727,#81728,#81729));
#18020=EDGE_LOOP('',(#81730,#81731,#81732,#81733));
#18021=EDGE_LOOP('',(#81734,#81735,#81736,#81737));
#18022=EDGE_LOOP('',(#81738,#81739,#81740,#81741));
#18023=EDGE_LOOP('',(#81742,#81743,#81744,#81745));
#18024=EDGE_LOOP('',(#81746,#81747,#81748,#81749,#81750));
#18025=EDGE_LOOP('',(#81751,#81752,#81753,#81754));
#18026=EDGE_LOOP('',(#81755,#81756,#81757,#81758));
#18027=EDGE_LOOP('',(#81759,#81760,#81761,#81762,#81763));
#18028=EDGE_LOOP('',(#81764,#81765,#81766,#81767));
#18029=EDGE_LOOP('',(#81768,#81769,#81770,#81771));
#18030=EDGE_LOOP('',(#81772,#81773,#81774,#81775));
#18031=EDGE_LOOP('',(#81776,#81777,#81778,#81779));
#18032=EDGE_LOOP('',(#81780,#81781,#81782,#81783,#81784));
#18033=EDGE_LOOP('',(#81785,#81786,#81787,#81788));
#18034=EDGE_LOOP('',(#81789,#81790,#81791,#81792));
#18035=EDGE_LOOP('',(#81793,#81794,#81795,#81796));
#18036=EDGE_LOOP('',(#81797,#81798,#81799,#81800));
#18037=EDGE_LOOP('',(#81801,#81802,#81803,#81804));
#18038=EDGE_LOOP('',(#81805,#81806,#81807,#81808));
#18039=EDGE_LOOP('',(#81809,#81810,#81811,#81812));
#18040=EDGE_LOOP('',(#81813,#81814,#81815,#81816));
#18041=EDGE_LOOP('',(#81817,#81818,#81819,#81820));
#18042=EDGE_LOOP('',(#81821,#81822,#81823,#81824));
#18043=EDGE_LOOP('',(#81825,#81826,#81827,#81828,#81829));
#18044=EDGE_LOOP('',(#81830,#81831,#81832,#81833));
#18045=EDGE_LOOP('',(#81834,#81835,#81836,#81837));
#18046=EDGE_LOOP('',(#81838,#81839,#81840,#81841));
#18047=EDGE_LOOP('',(#81842,#81843,#81844,#81845));
#18048=EDGE_LOOP('',(#81846,#81847,#81848,#81849));
#18049=EDGE_LOOP('',(#81850,#81851,#81852,#81853));
#18050=EDGE_LOOP('',(#81854,#81855,#81856,#81857));
#18051=EDGE_LOOP('',(#81858,#81859,#81860,#81861));
#18052=EDGE_LOOP('',(#81862,#81863,#81864,#81865,#81866));
#18053=EDGE_LOOP('',(#81867,#81868,#81869,#81870));
#18054=EDGE_LOOP('',(#81871,#81872,#81873,#81874));
#18055=EDGE_LOOP('',(#81875,#81876,#81877,#81878,#81879));
#18056=EDGE_LOOP('',(#81880,#81881,#81882,#81883));
#18057=EDGE_LOOP('',(#81884,#81885,#81886,#81887));
#18058=EDGE_LOOP('',(#81888,#81889,#81890,#81891));
#18059=EDGE_LOOP('',(#81892,#81893,#81894,#81895));
#18060=EDGE_LOOP('',(#81896,#81897,#81898,#81899,#81900));
#18061=EDGE_LOOP('',(#81901,#81902,#81903,#81904));
#18062=EDGE_LOOP('',(#81905,#81906,#81907,#81908));
#18063=EDGE_LOOP('',(#81909,#81910,#81911,#81912));
#18064=EDGE_LOOP('',(#81913,#81914,#81915,#81916));
#18065=EDGE_LOOP('',(#81917,#81918,#81919,#81920));
#18066=EDGE_LOOP('',(#81921,#81922,#81923,#81924));
#18067=EDGE_LOOP('',(#81925,#81926,#81927,#81928));
#18068=EDGE_LOOP('',(#81929,#81930,#81931,#81932));
#18069=EDGE_LOOP('',(#81933,#81934,#81935,#81936));
#18070=EDGE_LOOP('',(#81937,#81938,#81939,#81940));
#18071=EDGE_LOOP('',(#81941,#81942,#81943,#81944,#81945));
#18072=EDGE_LOOP('',(#81946,#81947,#81948,#81949));
#18073=EDGE_LOOP('',(#81950,#81951,#81952,#81953));
#18074=EDGE_LOOP('',(#81954,#81955,#81956,#81957));
#18075=EDGE_LOOP('',(#81958,#81959,#81960,#81961));
#18076=EDGE_LOOP('',(#81962,#81963,#81964,#81965));
#18077=EDGE_LOOP('',(#81966,#81967,#81968,#81969));
#18078=EDGE_LOOP('',(#81970,#81971,#81972,#81973));
#18079=EDGE_LOOP('',(#81974,#81975,#81976,#81977));
#18080=EDGE_LOOP('',(#81978,#81979,#81980,#81981,#81982));
#18081=EDGE_LOOP('',(#81983,#81984,#81985,#81986));
#18082=EDGE_LOOP('',(#81987,#81988,#81989,#81990));
#18083=EDGE_LOOP('',(#81991,#81992,#81993,#81994,#81995));
#18084=EDGE_LOOP('',(#81996,#81997,#81998,#81999));
#18085=EDGE_LOOP('',(#82000,#82001,#82002,#82003));
#18086=EDGE_LOOP('',(#82004,#82005,#82006,#82007));
#18087=EDGE_LOOP('',(#82008,#82009,#82010,#82011));
#18088=EDGE_LOOP('',(#82012,#82013,#82014,#82015,#82016));
#18089=EDGE_LOOP('',(#82017,#82018,#82019,#82020));
#18090=EDGE_LOOP('',(#82021,#82022,#82023,#82024));
#18091=EDGE_LOOP('',(#82025,#82026,#82027,#82028));
#18092=EDGE_LOOP('',(#82029,#82030,#82031,#82032));
#18093=EDGE_LOOP('',(#82033,#82034,#82035,#82036));
#18094=EDGE_LOOP('',(#82037,#82038,#82039,#82040));
#18095=EDGE_LOOP('',(#82041,#82042,#82043,#82044));
#18096=EDGE_LOOP('',(#82045,#82046,#82047,#82048));
#18097=EDGE_LOOP('',(#82049,#82050,#82051,#82052));
#18098=EDGE_LOOP('',(#82053,#82054,#82055,#82056));
#18099=EDGE_LOOP('',(#82057,#82058,#82059,#82060,#82061));
#18100=EDGE_LOOP('',(#82062,#82063,#82064,#82065));
#18101=EDGE_LOOP('',(#82066,#82067,#82068,#82069));
#18102=EDGE_LOOP('',(#82070,#82071,#82072,#82073));
#18103=EDGE_LOOP('',(#82074,#82075,#82076,#82077));
#18104=EDGE_LOOP('',(#82078,#82079,#82080,#82081));
#18105=EDGE_LOOP('',(#82082,#82083,#82084,#82085));
#18106=EDGE_LOOP('',(#82086,#82087,#82088,#82089));
#18107=EDGE_LOOP('',(#82090,#82091,#82092,#82093));
#18108=EDGE_LOOP('',(#82094,#82095,#82096,#82097,#82098));
#18109=EDGE_LOOP('',(#82099,#82100,#82101,#82102));
#18110=EDGE_LOOP('',(#82103,#82104,#82105,#82106));
#18111=EDGE_LOOP('',(#82107,#82108,#82109,#82110,#82111));
#18112=EDGE_LOOP('',(#82112,#82113,#82114,#82115));
#18113=EDGE_LOOP('',(#82116,#82117,#82118,#82119));
#18114=EDGE_LOOP('',(#82120,#82121,#82122,#82123));
#18115=EDGE_LOOP('',(#82124,#82125,#82126,#82127));
#18116=EDGE_LOOP('',(#82128,#82129,#82130,#82131,#82132));
#18117=EDGE_LOOP('',(#82133,#82134,#82135,#82136));
#18118=EDGE_LOOP('',(#82137,#82138,#82139,#82140));
#18119=EDGE_LOOP('',(#82141,#82142,#82143,#82144));
#18120=EDGE_LOOP('',(#82145,#82146,#82147,#82148));
#18121=EDGE_LOOP('',(#82149,#82150,#82151,#82152));
#18122=EDGE_LOOP('',(#82153,#82154,#82155,#82156));
#18123=EDGE_LOOP('',(#82157,#82158,#82159,#82160));
#18124=EDGE_LOOP('',(#82161,#82162,#82163,#82164));
#18125=EDGE_LOOP('',(#82165,#82166,#82167,#82168));
#18126=EDGE_LOOP('',(#82169,#82170,#82171,#82172));
#18127=EDGE_LOOP('',(#82173,#82174,#82175,#82176,#82177));
#18128=EDGE_LOOP('',(#82178,#82179,#82180,#82181));
#18129=EDGE_LOOP('',(#82182,#82183,#82184,#82185));
#18130=EDGE_LOOP('',(#82186,#82187,#82188,#82189));
#18131=EDGE_LOOP('',(#82190,#82191,#82192,#82193));
#18132=EDGE_LOOP('',(#82194,#82195,#82196,#82197));
#18133=EDGE_LOOP('',(#82198,#82199,#82200,#82201));
#18134=EDGE_LOOP('',(#82202,#82203,#82204,#82205));
#18135=EDGE_LOOP('',(#82206,#82207,#82208,#82209));
#18136=EDGE_LOOP('',(#82210,#82211,#82212,#82213,#82214));
#18137=EDGE_LOOP('',(#82215,#82216,#82217,#82218));
#18138=EDGE_LOOP('',(#82219,#82220,#82221,#82222));
#18139=EDGE_LOOP('',(#82223,#82224,#82225,#82226,#82227));
#18140=EDGE_LOOP('',(#82228,#82229,#82230,#82231));
#18141=EDGE_LOOP('',(#82232,#82233,#82234,#82235));
#18142=EDGE_LOOP('',(#82236,#82237,#82238,#82239));
#18143=EDGE_LOOP('',(#82240,#82241,#82242,#82243));
#18144=EDGE_LOOP('',(#82244,#82245,#82246,#82247,#82248));
#18145=EDGE_LOOP('',(#82249,#82250,#82251,#82252));
#18146=EDGE_LOOP('',(#82253,#82254,#82255,#82256));
#18147=EDGE_LOOP('',(#82257,#82258,#82259,#82260));
#18148=EDGE_LOOP('',(#82261,#82262,#82263,#82264));
#18149=EDGE_LOOP('',(#82265,#82266,#82267,#82268));
#18150=EDGE_LOOP('',(#82269,#82270,#82271,#82272));
#18151=EDGE_LOOP('',(#82273,#82274,#82275,#82276));
#18152=EDGE_LOOP('',(#82277,#82278,#82279,#82280));
#18153=EDGE_LOOP('',(#82281,#82282,#82283,#82284));
#18154=EDGE_LOOP('',(#82285,#82286,#82287,#82288));
#18155=EDGE_LOOP('',(#82289,#82290,#82291,#82292,#82293));
#18156=EDGE_LOOP('',(#82294,#82295,#82296,#82297));
#18157=EDGE_LOOP('',(#82298,#82299,#82300,#82301));
#18158=EDGE_LOOP('',(#82302,#82303,#82304,#82305));
#18159=EDGE_LOOP('',(#82306,#82307,#82308,#82309));
#18160=EDGE_LOOP('',(#82310,#82311,#82312,#82313));
#18161=EDGE_LOOP('',(#82314,#82315,#82316,#82317));
#18162=EDGE_LOOP('',(#82318,#82319,#82320,#82321));
#18163=EDGE_LOOP('',(#82322,#82323,#82324,#82325));
#18164=EDGE_LOOP('',(#82326,#82327,#82328,#82329,#82330));
#18165=EDGE_LOOP('',(#82331,#82332,#82333,#82334));
#18166=EDGE_LOOP('',(#82335,#82336,#82337,#82338));
#18167=EDGE_LOOP('',(#82339,#82340,#82341,#82342,#82343));
#18168=EDGE_LOOP('',(#82344,#82345,#82346,#82347));
#18169=EDGE_LOOP('',(#82348,#82349,#82350,#82351));
#18170=EDGE_LOOP('',(#82352,#82353,#82354,#82355));
#18171=EDGE_LOOP('',(#82356,#82357,#82358,#82359));
#18172=EDGE_LOOP('',(#82360,#82361,#82362,#82363,#82364));
#18173=EDGE_LOOP('',(#82365,#82366,#82367,#82368));
#18174=EDGE_LOOP('',(#82369,#82370,#82371,#82372));
#18175=EDGE_LOOP('',(#82373,#82374,#82375,#82376));
#18176=EDGE_LOOP('',(#82377,#82378,#82379,#82380));
#18177=EDGE_LOOP('',(#82381,#82382,#82383,#82384));
#18178=EDGE_LOOP('',(#82385,#82386,#82387,#82388));
#18179=EDGE_LOOP('',(#82389,#82390,#82391,#82392));
#18180=EDGE_LOOP('',(#82393,#82394,#82395,#82396));
#18181=EDGE_LOOP('',(#82397,#82398,#82399,#82400,#82401));
#18182=EDGE_LOOP('',(#82402,#82403,#82404,#82405));
#18183=EDGE_LOOP('',(#82406,#82407,#82408,#82409));
#18184=EDGE_LOOP('',(#82410,#82411,#82412,#82413));
#18185=EDGE_LOOP('',(#82414,#82415,#82416,#82417));
#18186=EDGE_LOOP('',(#82418,#82419,#82420,#82421));
#18187=EDGE_LOOP('',(#82422,#82423,#82424,#82425));
#18188=EDGE_LOOP('',(#82426,#82427,#82428,#82429));
#18189=EDGE_LOOP('',(#82430,#82431,#82432,#82433));
#18190=EDGE_LOOP('',(#82434,#82435,#82436,#82437,#82438));
#18191=EDGE_LOOP('',(#82439,#82440,#82441,#82442));
#18192=EDGE_LOOP('',(#82443,#82444,#82445,#82446));
#18193=EDGE_LOOP('',(#82447,#82448,#82449,#82450,#82451));
#18194=EDGE_LOOP('',(#82452,#82453,#82454,#82455));
#18195=EDGE_LOOP('',(#82456,#82457,#82458,#82459));
#18196=EDGE_LOOP('',(#82460,#82461,#82462,#82463));
#18197=EDGE_LOOP('',(#82464,#82465,#82466,#82467));
#18198=EDGE_LOOP('',(#82468,#82469,#82470,#82471,#82472));
#18199=EDGE_LOOP('',(#82473,#82474,#82475,#82476));
#18200=EDGE_LOOP('',(#82477,#82478,#82479,#82480));
#18201=EDGE_LOOP('',(#82481,#82482,#82483,#82484));
#18202=EDGE_LOOP('',(#82485,#82486,#82487,#82488));
#18203=EDGE_LOOP('',(#82489,#82490,#82491,#82492));
#18204=EDGE_LOOP('',(#82493,#82494,#82495,#82496));
#18205=EDGE_LOOP('',(#82497,#82498,#82499,#82500));
#18206=EDGE_LOOP('',(#82501,#82502,#82503,#82504));
#18207=EDGE_LOOP('',(#82505,#82506,#82507,#82508));
#18208=EDGE_LOOP('',(#82509,#82510,#82511,#82512));
#18209=EDGE_LOOP('',(#82513,#82514,#82515,#82516,#82517));
#18210=EDGE_LOOP('',(#82518,#82519,#82520,#82521));
#18211=EDGE_LOOP('',(#82522,#82523,#82524,#82525));
#18212=EDGE_LOOP('',(#82526,#82527,#82528,#82529));
#18213=EDGE_LOOP('',(#82530,#82531,#82532,#82533));
#18214=EDGE_LOOP('',(#82534,#82535,#82536,#82537));
#18215=EDGE_LOOP('',(#82538,#82539,#82540,#82541));
#18216=EDGE_LOOP('',(#82542,#82543,#82544,#82545));
#18217=EDGE_LOOP('',(#82546,#82547,#82548,#82549));
#18218=EDGE_LOOP('',(#82550,#82551,#82552,#82553,#82554));
#18219=EDGE_LOOP('',(#82555,#82556,#82557,#82558));
#18220=EDGE_LOOP('',(#82559,#82560,#82561,#82562));
#18221=EDGE_LOOP('',(#82563,#82564,#82565,#82566,#82567));
#18222=EDGE_LOOP('',(#82568,#82569,#82570,#82571));
#18223=EDGE_LOOP('',(#82572,#82573,#82574,#82575));
#18224=EDGE_LOOP('',(#82576,#82577,#82578,#82579));
#18225=EDGE_LOOP('',(#82580,#82581,#82582,#82583));
#18226=EDGE_LOOP('',(#82584,#82585,#82586,#82587,#82588));
#18227=EDGE_LOOP('',(#82589,#82590,#82591,#82592));
#18228=EDGE_LOOP('',(#82593,#82594,#82595,#82596));
#18229=EDGE_LOOP('',(#82597,#82598,#82599,#82600));
#18230=EDGE_LOOP('',(#82601,#82602,#82603,#82604));
#18231=EDGE_LOOP('',(#82605,#82606,#82607,#82608));
#18232=EDGE_LOOP('',(#82609,#82610,#82611,#82612));
#18233=EDGE_LOOP('',(#82613,#82614,#82615,#82616));
#18234=EDGE_LOOP('',(#82617,#82618,#82619,#82620));
#18235=EDGE_LOOP('',(#82621,#82622,#82623,#82624));
#18236=EDGE_LOOP('',(#82625,#82626,#82627,#82628));
#18237=EDGE_LOOP('',(#82629,#82630,#82631,#82632,#82633));
#18238=EDGE_LOOP('',(#82634,#82635,#82636,#82637));
#18239=EDGE_LOOP('',(#82638,#82639,#82640,#82641));
#18240=EDGE_LOOP('',(#82642,#82643,#82644,#82645));
#18241=EDGE_LOOP('',(#82646,#82647,#82648,#82649));
#18242=EDGE_LOOP('',(#82650,#82651,#82652,#82653));
#18243=EDGE_LOOP('',(#82654,#82655,#82656,#82657));
#18244=EDGE_LOOP('',(#82658,#82659,#82660,#82661));
#18245=EDGE_LOOP('',(#82662,#82663,#82664,#82665));
#18246=EDGE_LOOP('',(#82666,#82667,#82668,#82669,#82670));
#18247=EDGE_LOOP('',(#82671,#82672,#82673,#82674));
#18248=EDGE_LOOP('',(#82675,#82676,#82677,#82678));
#18249=EDGE_LOOP('',(#82679,#82680,#82681,#82682,#82683));
#18250=EDGE_LOOP('',(#82684,#82685,#82686,#82687));
#18251=EDGE_LOOP('',(#82688,#82689,#82690,#82691));
#18252=EDGE_LOOP('',(#82692,#82693,#82694,#82695));
#18253=EDGE_LOOP('',(#82696,#82697,#82698,#82699));
#18254=EDGE_LOOP('',(#82700,#82701,#82702,#82703,#82704));
#18255=EDGE_LOOP('',(#82705,#82706,#82707,#82708));
#18256=EDGE_LOOP('',(#82709,#82710,#82711,#82712));
#18257=EDGE_LOOP('',(#82713,#82714,#82715,#82716));
#18258=EDGE_LOOP('',(#82717,#82718,#82719,#82720));
#18259=EDGE_LOOP('',(#82721,#82722,#82723,#82724));
#18260=EDGE_LOOP('',(#82725,#82726,#82727,#82728));
#18261=EDGE_LOOP('',(#82729,#82730,#82731,#82732));
#18262=EDGE_LOOP('',(#82733,#82734,#82735,#82736));
#18263=EDGE_LOOP('',(#82737,#82738,#82739,#82740));
#18264=EDGE_LOOP('',(#82741,#82742,#82743,#82744));
#18265=EDGE_LOOP('',(#82745,#82746,#82747,#82748,#82749));
#18266=EDGE_LOOP('',(#82750,#82751,#82752,#82753));
#18267=EDGE_LOOP('',(#82754,#82755,#82756,#82757));
#18268=EDGE_LOOP('',(#82758,#82759,#82760,#82761));
#18269=EDGE_LOOP('',(#82762,#82763,#82764,#82765));
#18270=EDGE_LOOP('',(#82766,#82767,#82768,#82769));
#18271=EDGE_LOOP('',(#82770,#82771,#82772,#82773));
#18272=EDGE_LOOP('',(#82774,#82775,#82776,#82777));
#18273=EDGE_LOOP('',(#82778,#82779,#82780,#82781));
#18274=EDGE_LOOP('',(#82782,#82783,#82784,#82785,#82786));
#18275=EDGE_LOOP('',(#82787,#82788,#82789,#82790));
#18276=EDGE_LOOP('',(#82791,#82792,#82793,#82794));
#18277=EDGE_LOOP('',(#82795,#82796,#82797,#82798,#82799));
#18278=EDGE_LOOP('',(#82800,#82801,#82802,#82803));
#18279=EDGE_LOOP('',(#82804,#82805,#82806,#82807));
#18280=EDGE_LOOP('',(#82808,#82809,#82810,#82811));
#18281=EDGE_LOOP('',(#82812,#82813,#82814,#82815));
#18282=EDGE_LOOP('',(#82816,#82817,#82818,#82819,#82820));
#18283=EDGE_LOOP('',(#82821,#82822,#82823,#82824));
#18284=EDGE_LOOP('',(#82825,#82826,#82827,#82828));
#18285=EDGE_LOOP('',(#82829,#82830,#82831,#82832));
#18286=EDGE_LOOP('',(#82833,#82834,#82835,#82836));
#18287=EDGE_LOOP('',(#82837,#82838,#82839,#82840));
#18288=EDGE_LOOP('',(#82841,#82842,#82843,#82844));
#18289=EDGE_LOOP('',(#82845,#82846,#82847,#82848));
#18290=EDGE_LOOP('',(#82849,#82850,#82851,#82852));
#18291=EDGE_LOOP('',(#82853,#82854,#82855,#82856));
#18292=EDGE_LOOP('',(#82857,#82858,#82859,#82860));
#18293=EDGE_LOOP('',(#82861,#82862,#82863,#82864,#82865));
#18294=EDGE_LOOP('',(#82866,#82867,#82868,#82869));
#18295=EDGE_LOOP('',(#82870,#82871,#82872,#82873));
#18296=EDGE_LOOP('',(#82874,#82875,#82876,#82877));
#18297=EDGE_LOOP('',(#82878,#82879,#82880,#82881));
#18298=EDGE_LOOP('',(#82882,#82883,#82884,#82885));
#18299=EDGE_LOOP('',(#82886,#82887,#82888,#82889));
#18300=EDGE_LOOP('',(#82890,#82891,#82892,#82893));
#18301=EDGE_LOOP('',(#82894,#82895,#82896,#82897));
#18302=EDGE_LOOP('',(#82898,#82899,#82900,#82901,#82902));
#18303=EDGE_LOOP('',(#82903,#82904,#82905,#82906));
#18304=EDGE_LOOP('',(#82907,#82908,#82909,#82910));
#18305=EDGE_LOOP('',(#82911,#82912,#82913,#82914,#82915));
#18306=EDGE_LOOP('',(#82916,#82917,#82918,#82919));
#18307=EDGE_LOOP('',(#82920,#82921,#82922,#82923));
#18308=EDGE_LOOP('',(#82924,#82925,#82926,#82927));
#18309=EDGE_LOOP('',(#82928,#82929,#82930,#82931));
#18310=EDGE_LOOP('',(#82932,#82933,#82934,#82935,#82936));
#18311=EDGE_LOOP('',(#82937,#82938,#82939,#82940));
#18312=EDGE_LOOP('',(#82941,#82942,#82943,#82944));
#18313=EDGE_LOOP('',(#82945,#82946,#82947,#82948));
#18314=EDGE_LOOP('',(#82949,#82950,#82951,#82952));
#18315=EDGE_LOOP('',(#82953,#82954,#82955,#82956));
#18316=EDGE_LOOP('',(#82957,#82958,#82959,#82960));
#18317=EDGE_LOOP('',(#82961,#82962,#82963,#82964));
#18318=EDGE_LOOP('',(#82965,#82966,#82967,#82968));
#18319=EDGE_LOOP('',(#82969,#82970,#82971,#82972));
#18320=EDGE_LOOP('',(#82973,#82974,#82975,#82976));
#18321=EDGE_LOOP('',(#82977,#82978,#82979,#82980,#82981));
#18322=EDGE_LOOP('',(#82982,#82983,#82984,#82985));
#18323=EDGE_LOOP('',(#82986,#82987,#82988,#82989));
#18324=EDGE_LOOP('',(#82990,#82991,#82992,#82993));
#18325=EDGE_LOOP('',(#82994,#82995,#82996,#82997));
#18326=EDGE_LOOP('',(#82998,#82999,#83000,#83001));
#18327=EDGE_LOOP('',(#83002,#83003,#83004,#83005));
#18328=EDGE_LOOP('',(#83006,#83007,#83008,#83009));
#18329=EDGE_LOOP('',(#83010,#83011,#83012,#83013));
#18330=EDGE_LOOP('',(#83014,#83015,#83016,#83017,#83018));
#18331=EDGE_LOOP('',(#83019,#83020,#83021,#83022));
#18332=EDGE_LOOP('',(#83023,#83024,#83025,#83026));
#18333=EDGE_LOOP('',(#83027,#83028,#83029,#83030,#83031));
#18334=EDGE_LOOP('',(#83032,#83033,#83034,#83035));
#18335=EDGE_LOOP('',(#83036,#83037,#83038,#83039));
#18336=EDGE_LOOP('',(#83040,#83041,#83042,#83043));
#18337=EDGE_LOOP('',(#83044,#83045,#83046,#83047));
#18338=EDGE_LOOP('',(#83048,#83049,#83050,#83051,#83052));
#18339=EDGE_LOOP('',(#83053,#83054,#83055,#83056));
#18340=EDGE_LOOP('',(#83057,#83058,#83059,#83060));
#18341=EDGE_LOOP('',(#83061,#83062,#83063,#83064));
#18342=EDGE_LOOP('',(#83065,#83066,#83067,#83068));
#18343=EDGE_LOOP('',(#83069,#83070,#83071,#83072));
#18344=EDGE_LOOP('',(#83073,#83074,#83075,#83076));
#18345=EDGE_LOOP('',(#83077,#83078,#83079,#83080));
#18346=EDGE_LOOP('',(#83081,#83082,#83083,#83084));
#18347=EDGE_LOOP('',(#83085,#83086,#83087,#83088));
#18348=EDGE_LOOP('',(#83089,#83090,#83091,#83092));
#18349=EDGE_LOOP('',(#83093,#83094,#83095,#83096,#83097));
#18350=EDGE_LOOP('',(#83098,#83099,#83100,#83101));
#18351=EDGE_LOOP('',(#83102,#83103,#83104,#83105));
#18352=EDGE_LOOP('',(#83106,#83107,#83108,#83109));
#18353=EDGE_LOOP('',(#83110,#83111,#83112,#83113));
#18354=EDGE_LOOP('',(#83114,#83115,#83116,#83117));
#18355=EDGE_LOOP('',(#83118,#83119,#83120,#83121));
#18356=EDGE_LOOP('',(#83122,#83123,#83124,#83125));
#18357=EDGE_LOOP('',(#83126,#83127,#83128,#83129));
#18358=EDGE_LOOP('',(#83130,#83131,#83132,#83133,#83134));
#18359=EDGE_LOOP('',(#83135,#83136,#83137,#83138));
#18360=EDGE_LOOP('',(#83139,#83140,#83141,#83142));
#18361=EDGE_LOOP('',(#83143,#83144,#83145,#83146,#83147));
#18362=EDGE_LOOP('',(#83148,#83149,#83150,#83151));
#18363=EDGE_LOOP('',(#83152,#83153,#83154,#83155));
#18364=EDGE_LOOP('',(#83156,#83157,#83158,#83159));
#18365=EDGE_LOOP('',(#83160,#83161,#83162,#83163));
#18366=EDGE_LOOP('',(#83164,#83165,#83166,#83167,#83168));
#18367=EDGE_LOOP('',(#83169,#83170,#83171,#83172));
#18368=EDGE_LOOP('',(#83173,#83174,#83175,#83176));
#18369=EDGE_LOOP('',(#83177,#83178,#83179,#83180));
#18370=EDGE_LOOP('',(#83181,#83182,#83183,#83184));
#18371=EDGE_LOOP('',(#83185,#83186,#83187,#83188));
#18372=EDGE_LOOP('',(#83189,#83190,#83191,#83192));
#18373=EDGE_LOOP('',(#83193,#83194,#83195,#83196));
#18374=EDGE_LOOP('',(#83197,#83198,#83199,#83200));
#18375=EDGE_LOOP('',(#83201,#83202,#83203,#83204));
#18376=EDGE_LOOP('',(#83205,#83206,#83207,#83208));
#18377=EDGE_LOOP('',(#83209,#83210,#83211,#83212,#83213));
#18378=EDGE_LOOP('',(#83214,#83215,#83216,#83217));
#18379=EDGE_LOOP('',(#83218,#83219,#83220,#83221));
#18380=EDGE_LOOP('',(#83222,#83223,#83224,#83225));
#18381=EDGE_LOOP('',(#83226,#83227,#83228,#83229));
#18382=EDGE_LOOP('',(#83230,#83231,#83232,#83233));
#18383=EDGE_LOOP('',(#83234,#83235,#83236,#83237));
#18384=EDGE_LOOP('',(#83238,#83239,#83240,#83241));
#18385=EDGE_LOOP('',(#83242,#83243,#83244,#83245));
#18386=EDGE_LOOP('',(#83246,#83247,#83248,#83249,#83250));
#18387=EDGE_LOOP('',(#83251,#83252,#83253,#83254));
#18388=EDGE_LOOP('',(#83255,#83256,#83257,#83258));
#18389=EDGE_LOOP('',(#83259,#83260,#83261,#83262,#83263));
#18390=EDGE_LOOP('',(#83264,#83265,#83266,#83267));
#18391=EDGE_LOOP('',(#83268,#83269,#83270,#83271));
#18392=EDGE_LOOP('',(#83272,#83273,#83274,#83275));
#18393=EDGE_LOOP('',(#83276,#83277,#83278,#83279));
#18394=EDGE_LOOP('',(#83280,#83281,#83282,#83283,#83284));
#18395=EDGE_LOOP('',(#83285,#83286,#83287,#83288));
#18396=EDGE_LOOP('',(#83289,#83290,#83291,#83292));
#18397=EDGE_LOOP('',(#83293,#83294,#83295,#83296));
#18398=EDGE_LOOP('',(#83297,#83298,#83299,#83300));
#18399=EDGE_LOOP('',(#83301,#83302,#83303,#83304));
#18400=EDGE_LOOP('',(#83305,#83306,#83307,#83308));
#18401=EDGE_LOOP('',(#83309,#83310,#83311,#83312));
#18402=EDGE_LOOP('',(#83313,#83314,#83315,#83316));
#18403=EDGE_LOOP('',(#83317,#83318,#83319,#83320));
#18404=EDGE_LOOP('',(#83321,#83322,#83323,#83324));
#18405=EDGE_LOOP('',(#83325,#83326,#83327,#83328,#83329));
#18406=EDGE_LOOP('',(#83330,#83331,#83332,#83333));
#18407=EDGE_LOOP('',(#83334,#83335,#83336,#83337));
#18408=EDGE_LOOP('',(#83338,#83339,#83340,#83341));
#18409=EDGE_LOOP('',(#83342,#83343,#83344,#83345));
#18410=EDGE_LOOP('',(#83346,#83347,#83348,#83349));
#18411=EDGE_LOOP('',(#83350,#83351,#83352,#83353));
#18412=EDGE_LOOP('',(#83354,#83355,#83356,#83357));
#18413=EDGE_LOOP('',(#83358,#83359,#83360,#83361));
#18414=EDGE_LOOP('',(#83362,#83363,#83364,#83365,#83366));
#18415=EDGE_LOOP('',(#83367,#83368,#83369,#83370));
#18416=EDGE_LOOP('',(#83371,#83372,#83373,#83374));
#18417=EDGE_LOOP('',(#83375,#83376,#83377,#83378,#83379));
#18418=EDGE_LOOP('',(#83380,#83381,#83382,#83383));
#18419=EDGE_LOOP('',(#83384,#83385,#83386,#83387));
#18420=EDGE_LOOP('',(#83388,#83389,#83390,#83391));
#18421=EDGE_LOOP('',(#83392,#83393,#83394,#83395));
#18422=EDGE_LOOP('',(#83396,#83397,#83398,#83399,#83400));
#18423=EDGE_LOOP('',(#83401,#83402,#83403,#83404));
#18424=EDGE_LOOP('',(#83405,#83406,#83407,#83408));
#18425=EDGE_LOOP('',(#83409,#83410,#83411,#83412));
#18426=EDGE_LOOP('',(#83413,#83414,#83415,#83416));
#18427=EDGE_LOOP('',(#83417,#83418,#83419,#83420));
#18428=EDGE_LOOP('',(#83421,#83422,#83423,#83424));
#18429=EDGE_LOOP('',(#83425,#83426,#83427,#83428));
#18430=EDGE_LOOP('',(#83429,#83430,#83431,#83432));
#18431=EDGE_LOOP('',(#83433,#83434,#83435,#83436));
#18432=EDGE_LOOP('',(#83437,#83438,#83439,#83440));
#18433=EDGE_LOOP('',(#83441,#83442,#83443,#83444,#83445));
#18434=EDGE_LOOP('',(#83446,#83447,#83448,#83449));
#18435=EDGE_LOOP('',(#83450,#83451,#83452,#83453));
#18436=EDGE_LOOP('',(#83454,#83455,#83456,#83457));
#18437=EDGE_LOOP('',(#83458,#83459,#83460,#83461));
#18438=EDGE_LOOP('',(#83462,#83463,#83464,#83465));
#18439=EDGE_LOOP('',(#83466,#83467,#83468,#83469));
#18440=EDGE_LOOP('',(#83470,#83471,#83472,#83473));
#18441=EDGE_LOOP('',(#83474,#83475,#83476,#83477));
#18442=EDGE_LOOP('',(#83478,#83479,#83480,#83481,#83482));
#18443=EDGE_LOOP('',(#83483,#83484,#83485,#83486));
#18444=EDGE_LOOP('',(#83487,#83488,#83489,#83490));
#18445=EDGE_LOOP('',(#83491,#83492,#83493,#83494,#83495));
#18446=EDGE_LOOP('',(#83496,#83497,#83498,#83499));
#18447=EDGE_LOOP('',(#83500,#83501,#83502,#83503));
#18448=EDGE_LOOP('',(#83504,#83505,#83506,#83507));
#18449=EDGE_LOOP('',(#83508,#83509,#83510,#83511));
#18450=EDGE_LOOP('',(#83512,#83513,#83514,#83515,#83516));
#18451=EDGE_LOOP('',(#83517,#83518,#83519,#83520));
#18452=EDGE_LOOP('',(#83521,#83522,#83523,#83524));
#18453=EDGE_LOOP('',(#83525,#83526,#83527,#83528));
#18454=EDGE_LOOP('',(#83529,#83530,#83531,#83532));
#18455=EDGE_LOOP('',(#83533,#83534,#83535,#83536));
#18456=EDGE_LOOP('',(#83537,#83538,#83539,#83540));
#18457=EDGE_LOOP('',(#83541,#83542,#83543,#83544));
#18458=EDGE_LOOP('',(#83545,#83546,#83547,#83548));
#18459=EDGE_LOOP('',(#83549,#83550,#83551,#83552));
#18460=EDGE_LOOP('',(#83553,#83554,#83555,#83556));
#18461=EDGE_LOOP('',(#83557,#83558,#83559,#83560,#83561));
#18462=EDGE_LOOP('',(#83562,#83563,#83564,#83565));
#18463=EDGE_LOOP('',(#83566,#83567,#83568,#83569));
#18464=EDGE_LOOP('',(#83570,#83571,#83572,#83573));
#18465=EDGE_LOOP('',(#83574,#83575,#83576,#83577));
#18466=EDGE_LOOP('',(#83578,#83579,#83580,#83581));
#18467=EDGE_LOOP('',(#83582,#83583,#83584,#83585));
#18468=EDGE_LOOP('',(#83586,#83587,#83588,#83589));
#18469=EDGE_LOOP('',(#83590,#83591,#83592,#83593));
#18470=EDGE_LOOP('',(#83594,#83595,#83596,#83597,#83598));
#18471=EDGE_LOOP('',(#83599,#83600,#83601,#83602));
#18472=EDGE_LOOP('',(#83603,#83604,#83605,#83606));
#18473=EDGE_LOOP('',(#83607,#83608,#83609,#83610,#83611));
#18474=EDGE_LOOP('',(#83612,#83613,#83614,#83615));
#18475=EDGE_LOOP('',(#83616,#83617,#83618,#83619));
#18476=EDGE_LOOP('',(#83620,#83621,#83622,#83623));
#18477=EDGE_LOOP('',(#83624,#83625,#83626,#83627));
#18478=EDGE_LOOP('',(#83628,#83629,#83630,#83631,#83632));
#18479=EDGE_LOOP('',(#83633,#83634,#83635,#83636));
#18480=EDGE_LOOP('',(#83637,#83638,#83639,#83640));
#18481=EDGE_LOOP('',(#83641,#83642,#83643,#83644));
#18482=EDGE_LOOP('',(#83645,#83646,#83647,#83648));
#18483=EDGE_LOOP('',(#83649,#83650,#83651,#83652));
#18484=EDGE_LOOP('',(#83653,#83654,#83655,#83656));
#18485=EDGE_LOOP('',(#83657,#83658,#83659,#83660));
#18486=EDGE_LOOP('',(#83661,#83662,#83663,#83664));
#18487=EDGE_LOOP('',(#83665,#83666,#83667,#83668));
#18488=EDGE_LOOP('',(#83669,#83670,#83671,#83672));
#18489=EDGE_LOOP('',(#83673,#83674,#83675,#83676,#83677));
#18490=EDGE_LOOP('',(#83678,#83679,#83680,#83681));
#18491=EDGE_LOOP('',(#83682,#83683,#83684,#83685));
#18492=EDGE_LOOP('',(#83686,#83687,#83688,#83689));
#18493=EDGE_LOOP('',(#83690,#83691,#83692,#83693));
#18494=EDGE_LOOP('',(#83694,#83695,#83696,#83697));
#18495=EDGE_LOOP('',(#83698,#83699,#83700,#83701));
#18496=EDGE_LOOP('',(#83702,#83703,#83704,#83705));
#18497=EDGE_LOOP('',(#83706,#83707,#83708,#83709));
#18498=EDGE_LOOP('',(#83710,#83711,#83712,#83713,#83714));
#18499=EDGE_LOOP('',(#83715,#83716,#83717,#83718));
#18500=EDGE_LOOP('',(#83719,#83720,#83721,#83722));
#18501=EDGE_LOOP('',(#83723,#83724,#83725,#83726,#83727));
#18502=EDGE_LOOP('',(#83728,#83729,#83730,#83731));
#18503=EDGE_LOOP('',(#83732,#83733,#83734,#83735));
#18504=EDGE_LOOP('',(#83736,#83737,#83738,#83739));
#18505=EDGE_LOOP('',(#83740,#83741,#83742,#83743));
#18506=EDGE_LOOP('',(#83744,#83745,#83746,#83747,#83748));
#18507=EDGE_LOOP('',(#83749,#83750,#83751,#83752));
#18508=EDGE_LOOP('',(#83753,#83754,#83755,#83756));
#18509=EDGE_LOOP('',(#83757,#83758,#83759,#83760));
#18510=EDGE_LOOP('',(#83761,#83762,#83763,#83764));
#18511=EDGE_LOOP('',(#83765,#83766,#83767,#83768));
#18512=EDGE_LOOP('',(#83769,#83770,#83771,#83772));
#18513=EDGE_LOOP('',(#83773,#83774,#83775,#83776));
#18514=EDGE_LOOP('',(#83777,#83778,#83779,#83780));
#18515=EDGE_LOOP('',(#83781,#83782,#83783,#83784));
#18516=EDGE_LOOP('',(#83785,#83786,#83787,#83788));
#18517=EDGE_LOOP('',(#83789,#83790,#83791,#83792,#83793));
#18518=EDGE_LOOP('',(#83794,#83795,#83796,#83797));
#18519=EDGE_LOOP('',(#83798,#83799,#83800,#83801));
#18520=EDGE_LOOP('',(#83802,#83803,#83804,#83805));
#18521=EDGE_LOOP('',(#83806,#83807,#83808,#83809));
#18522=EDGE_LOOP('',(#83810,#83811,#83812,#83813));
#18523=EDGE_LOOP('',(#83814,#83815,#83816,#83817));
#18524=EDGE_LOOP('',(#83818,#83819,#83820,#83821));
#18525=EDGE_LOOP('',(#83822,#83823,#83824,#83825));
#18526=EDGE_LOOP('',(#83826,#83827,#83828,#83829,#83830));
#18527=EDGE_LOOP('',(#83831,#83832,#83833,#83834));
#18528=EDGE_LOOP('',(#83835,#83836,#83837,#83838));
#18529=EDGE_LOOP('',(#83839,#83840,#83841,#83842,#83843));
#18530=EDGE_LOOP('',(#83844,#83845,#83846,#83847));
#18531=EDGE_LOOP('',(#83848,#83849,#83850,#83851));
#18532=EDGE_LOOP('',(#83852,#83853,#83854,#83855));
#18533=EDGE_LOOP('',(#83856,#83857,#83858,#83859));
#18534=EDGE_LOOP('',(#83860,#83861,#83862,#83863,#83864));
#18535=EDGE_LOOP('',(#83865,#83866,#83867,#83868));
#18536=EDGE_LOOP('',(#83869,#83870,#83871,#83872));
#18537=EDGE_LOOP('',(#83873,#83874,#83875,#83876));
#18538=EDGE_LOOP('',(#83877,#83878,#83879,#83880));
#18539=EDGE_LOOP('',(#83881,#83882,#83883,#83884));
#18540=EDGE_LOOP('',(#83885,#83886,#83887,#83888));
#18541=EDGE_LOOP('',(#83889,#83890,#83891,#83892));
#18542=EDGE_LOOP('',(#83893,#83894,#83895,#83896));
#18543=EDGE_LOOP('',(#83897,#83898,#83899,#83900));
#18544=EDGE_LOOP('',(#83901,#83902,#83903,#83904));
#18545=EDGE_LOOP('',(#83905,#83906,#83907,#83908,#83909));
#18546=EDGE_LOOP('',(#83910,#83911,#83912,#83913));
#18547=EDGE_LOOP('',(#83914,#83915,#83916,#83917));
#18548=EDGE_LOOP('',(#83918,#83919,#83920,#83921));
#18549=EDGE_LOOP('',(#83922,#83923,#83924,#83925));
#18550=EDGE_LOOP('',(#83926,#83927,#83928,#83929));
#18551=EDGE_LOOP('',(#83930,#83931,#83932,#83933));
#18552=EDGE_LOOP('',(#83934,#83935,#83936,#83937));
#18553=EDGE_LOOP('',(#83938,#83939,#83940,#83941));
#18554=EDGE_LOOP('',(#83942,#83943,#83944,#83945,#83946));
#18555=EDGE_LOOP('',(#83947,#83948,#83949,#83950));
#18556=EDGE_LOOP('',(#83951,#83952,#83953,#83954));
#18557=EDGE_LOOP('',(#83955,#83956,#83957,#83958,#83959));
#18558=EDGE_LOOP('',(#83960,#83961,#83962,#83963));
#18559=EDGE_LOOP('',(#83964,#83965,#83966,#83967));
#18560=EDGE_LOOP('',(#83968,#83969,#83970,#83971));
#18561=EDGE_LOOP('',(#83972,#83973,#83974,#83975));
#18562=EDGE_LOOP('',(#83976,#83977,#83978,#83979,#83980));
#18563=EDGE_LOOP('',(#83981,#83982,#83983,#83984));
#18564=EDGE_LOOP('',(#83985,#83986,#83987,#83988));
#18565=EDGE_LOOP('',(#83989,#83990,#83991,#83992));
#18566=EDGE_LOOP('',(#83993,#83994,#83995,#83996));
#18567=EDGE_LOOP('',(#83997,#83998,#83999,#84000));
#18568=EDGE_LOOP('',(#84001,#84002,#84003,#84004));
#18569=EDGE_LOOP('',(#84005,#84006,#84007,#84008));
#18570=EDGE_LOOP('',(#84009,#84010,#84011,#84012));
#18571=EDGE_LOOP('',(#84013,#84014,#84015,#84016));
#18572=EDGE_LOOP('',(#84017,#84018,#84019,#84020));
#18573=EDGE_LOOP('',(#84021,#84022,#84023,#84024,#84025));
#18574=EDGE_LOOP('',(#84026,#84027,#84028,#84029));
#18575=EDGE_LOOP('',(#84030,#84031,#84032,#84033));
#18576=EDGE_LOOP('',(#84034,#84035,#84036,#84037));
#18577=EDGE_LOOP('',(#84038,#84039,#84040,#84041));
#18578=EDGE_LOOP('',(#84042,#84043,#84044,#84045));
#18579=EDGE_LOOP('',(#84046,#84047,#84048,#84049));
#18580=EDGE_LOOP('',(#84050,#84051,#84052,#84053));
#18581=EDGE_LOOP('',(#84054,#84055,#84056,#84057));
#18582=EDGE_LOOP('',(#84058,#84059,#84060,#84061,#84062));
#18583=EDGE_LOOP('',(#84063,#84064,#84065,#84066));
#18584=EDGE_LOOP('',(#84067,#84068,#84069,#84070));
#18585=EDGE_LOOP('',(#84071,#84072,#84073,#84074,#84075));
#18586=EDGE_LOOP('',(#84076,#84077,#84078,#84079));
#18587=EDGE_LOOP('',(#84080,#84081,#84082,#84083));
#18588=EDGE_LOOP('',(#84084,#84085,#84086,#84087));
#18589=EDGE_LOOP('',(#84088,#84089,#84090,#84091));
#18590=EDGE_LOOP('',(#84092,#84093,#84094,#84095,#84096));
#18591=EDGE_LOOP('',(#84097,#84098,#84099,#84100));
#18592=EDGE_LOOP('',(#84101,#84102,#84103,#84104));
#18593=EDGE_LOOP('',(#84105,#84106,#84107,#84108));
#18594=EDGE_LOOP('',(#84109,#84110,#84111,#84112));
#18595=EDGE_LOOP('',(#84113,#84114,#84115,#84116));
#18596=EDGE_LOOP('',(#84117,#84118,#84119,#84120));
#18597=EDGE_LOOP('',(#84121,#84122,#84123,#84124));
#18598=EDGE_LOOP('',(#84125,#84126,#84127,#84128));
#18599=EDGE_LOOP('',(#84129,#84130,#84131,#84132,#84133));
#18600=EDGE_LOOP('',(#84134,#84135,#84136,#84137));
#18601=EDGE_LOOP('',(#84138,#84139,#84140,#84141));
#18602=EDGE_LOOP('',(#84142,#84143,#84144,#84145));
#18603=EDGE_LOOP('',(#84146,#84147,#84148,#84149));
#18604=EDGE_LOOP('',(#84150,#84151,#84152,#84153));
#18605=EDGE_LOOP('',(#84154,#84155,#84156,#84157));
#18606=EDGE_LOOP('',(#84158,#84159,#84160,#84161));
#18607=EDGE_LOOP('',(#84162,#84163,#84164,#84165));
#18608=EDGE_LOOP('',(#84166,#84167,#84168,#84169,#84170));
#18609=EDGE_LOOP('',(#84171,#84172,#84173,#84174));
#18610=EDGE_LOOP('',(#84175,#84176,#84177,#84178));
#18611=EDGE_LOOP('',(#84179,#84180,#84181,#84182,#84183));
#18612=EDGE_LOOP('',(#84184,#84185,#84186,#84187));
#18613=EDGE_LOOP('',(#84188,#84189,#84190,#84191));
#18614=EDGE_LOOP('',(#84192,#84193,#84194,#84195));
#18615=EDGE_LOOP('',(#84196,#84197,#84198,#84199));
#18616=EDGE_LOOP('',(#84200,#84201,#84202,#84203,#84204));
#18617=EDGE_LOOP('',(#84205,#84206,#84207,#84208));
#18618=EDGE_LOOP('',(#84209,#84210,#84211,#84212));
#18619=EDGE_LOOP('',(#84213,#84214,#84215,#84216));
#18620=EDGE_LOOP('',(#84217,#84218,#84219,#84220));
#18621=EDGE_LOOP('',(#84221,#84222,#84223,#84224));
#18622=EDGE_LOOP('',(#84225,#84226,#84227,#84228));
#18623=EDGE_LOOP('',(#84229,#84230,#84231,#84232));
#18624=EDGE_LOOP('',(#84233,#84234,#84235,#84236));
#18625=EDGE_LOOP('',(#84237,#84238,#84239,#84240));
#18626=EDGE_LOOP('',(#84241,#84242,#84243,#84244));
#18627=EDGE_LOOP('',(#84245,#84246,#84247,#84248,#84249));
#18628=EDGE_LOOP('',(#84250,#84251,#84252,#84253));
#18629=EDGE_LOOP('',(#84254,#84255,#84256,#84257));
#18630=EDGE_LOOP('',(#84258,#84259,#84260,#84261));
#18631=EDGE_LOOP('',(#84262,#84263,#84264,#84265));
#18632=EDGE_LOOP('',(#84266,#84267,#84268,#84269));
#18633=EDGE_LOOP('',(#84270,#84271,#84272,#84273));
#18634=EDGE_LOOP('',(#84274,#84275,#84276,#84277));
#18635=EDGE_LOOP('',(#84278,#84279,#84280,#84281));
#18636=EDGE_LOOP('',(#84282,#84283,#84284,#84285,#84286));
#18637=EDGE_LOOP('',(#84287,#84288,#84289,#84290));
#18638=EDGE_LOOP('',(#84291,#84292,#84293,#84294));
#18639=EDGE_LOOP('',(#84295,#84296,#84297,#84298,#84299));
#18640=EDGE_LOOP('',(#84300,#84301,#84302,#84303));
#18641=EDGE_LOOP('',(#84304,#84305,#84306,#84307));
#18642=EDGE_LOOP('',(#84308,#84309,#84310,#84311));
#18643=EDGE_LOOP('',(#84312,#84313,#84314,#84315));
#18644=EDGE_LOOP('',(#84316,#84317,#84318,#84319,#84320));
#18645=EDGE_LOOP('',(#84321,#84322,#84323,#84324));
#18646=EDGE_LOOP('',(#84325,#84326,#84327,#84328));
#18647=EDGE_LOOP('',(#84329,#84330,#84331,#84332));
#18648=EDGE_LOOP('',(#84333,#84334,#84335,#84336));
#18649=EDGE_LOOP('',(#84337,#84338,#84339,#84340));
#18650=EDGE_LOOP('',(#84341,#84342,#84343,#84344));
#18651=EDGE_LOOP('',(#84345,#84346,#84347,#84348));
#18652=EDGE_LOOP('',(#84349,#84350,#84351,#84352));
#18653=EDGE_LOOP('',(#84353,#84354,#84355,#84356));
#18654=EDGE_LOOP('',(#84357,#84358,#84359,#84360));
#18655=EDGE_LOOP('',(#84361,#84362,#84363,#84364,#84365));
#18656=EDGE_LOOP('',(#84366,#84367,#84368,#84369));
#18657=EDGE_LOOP('',(#84370,#84371,#84372,#84373));
#18658=EDGE_LOOP('',(#84374,#84375,#84376,#84377));
#18659=EDGE_LOOP('',(#84378,#84379,#84380,#84381));
#18660=EDGE_LOOP('',(#84382,#84383,#84384,#84385));
#18661=EDGE_LOOP('',(#84386,#84387,#84388,#84389));
#18662=EDGE_LOOP('',(#84390,#84391,#84392,#84393));
#18663=EDGE_LOOP('',(#84394,#84395,#84396,#84397));
#18664=EDGE_LOOP('',(#84398,#84399,#84400,#84401,#84402));
#18665=EDGE_LOOP('',(#84403,#84404,#84405,#84406));
#18666=EDGE_LOOP('',(#84407,#84408,#84409,#84410));
#18667=EDGE_LOOP('',(#84411,#84412,#84413,#84414,#84415));
#18668=EDGE_LOOP('',(#84416,#84417,#84418,#84419));
#18669=EDGE_LOOP('',(#84420,#84421,#84422,#84423));
#18670=EDGE_LOOP('',(#84424,#84425,#84426,#84427));
#18671=EDGE_LOOP('',(#84428,#84429,#84430,#84431));
#18672=EDGE_LOOP('',(#84432,#84433,#84434,#84435,#84436));
#18673=EDGE_LOOP('',(#84437,#84438,#84439,#84440));
#18674=EDGE_LOOP('',(#84441,#84442,#84443,#84444));
#18675=EDGE_LOOP('',(#84445,#84446,#84447,#84448));
#18676=EDGE_LOOP('',(#84449,#84450,#84451,#84452));
#18677=EDGE_LOOP('',(#84453,#84454,#84455,#84456));
#18678=EDGE_LOOP('',(#84457,#84458,#84459,#84460));
#18679=EDGE_LOOP('',(#84461,#84462,#84463,#84464));
#18680=EDGE_LOOP('',(#84465,#84466,#84467,#84468));
#18681=EDGE_LOOP('',(#84469,#84470,#84471,#84472));
#18682=EDGE_LOOP('',(#84473,#84474,#84475,#84476));
#18683=EDGE_LOOP('',(#84477,#84478,#84479,#84480,#84481));
#18684=EDGE_LOOP('',(#84482,#84483,#84484,#84485));
#18685=EDGE_LOOP('',(#84486,#84487,#84488,#84489));
#18686=EDGE_LOOP('',(#84490,#84491,#84492,#84493));
#18687=EDGE_LOOP('',(#84494,#84495,#84496,#84497));
#18688=EDGE_LOOP('',(#84498,#84499,#84500,#84501));
#18689=EDGE_LOOP('',(#84502,#84503,#84504,#84505));
#18690=EDGE_LOOP('',(#84506,#84507,#84508,#84509));
#18691=EDGE_LOOP('',(#84510,#84511,#84512,#84513));
#18692=EDGE_LOOP('',(#84514,#84515,#84516,#84517,#84518));
#18693=EDGE_LOOP('',(#84519,#84520,#84521,#84522));
#18694=EDGE_LOOP('',(#84523,#84524,#84525,#84526));
#18695=EDGE_LOOP('',(#84527,#84528,#84529,#84530,#84531));
#18696=EDGE_LOOP('',(#84532,#84533,#84534,#84535));
#18697=EDGE_LOOP('',(#84536,#84537,#84538,#84539));
#18698=EDGE_LOOP('',(#84540,#84541,#84542,#84543));
#18699=EDGE_LOOP('',(#84544,#84545,#84546,#84547));
#18700=EDGE_LOOP('',(#84548,#84549,#84550,#84551,#84552));
#18701=EDGE_LOOP('',(#84553,#84554,#84555,#84556));
#18702=EDGE_LOOP('',(#84557,#84558,#84559,#84560));
#18703=EDGE_LOOP('',(#84561,#84562,#84563,#84564));
#18704=EDGE_LOOP('',(#84565,#84566,#84567,#84568));
#18705=EDGE_LOOP('',(#84569,#84570,#84571,#84572));
#18706=EDGE_LOOP('',(#84573,#84574,#84575,#84576));
#18707=EDGE_LOOP('',(#84577,#84578,#84579,#84580));
#18708=EDGE_LOOP('',(#84581,#84582,#84583,#84584));
#18709=EDGE_LOOP('',(#84585,#84586,#84587,#84588));
#18710=EDGE_LOOP('',(#84589,#84590,#84591,#84592));
#18711=EDGE_LOOP('',(#84593,#84594,#84595,#84596,#84597));
#18712=EDGE_LOOP('',(#84598,#84599,#84600,#84601));
#18713=EDGE_LOOP('',(#84602,#84603,#84604,#84605));
#18714=EDGE_LOOP('',(#84606,#84607,#84608,#84609));
#18715=EDGE_LOOP('',(#84610,#84611,#84612,#84613));
#18716=EDGE_LOOP('',(#84614,#84615,#84616,#84617));
#18717=EDGE_LOOP('',(#84618,#84619,#84620,#84621));
#18718=EDGE_LOOP('',(#84622,#84623,#84624,#84625));
#18719=EDGE_LOOP('',(#84626,#84627,#84628,#84629));
#18720=EDGE_LOOP('',(#84630,#84631,#84632,#84633,#84634));
#18721=EDGE_LOOP('',(#84635,#84636,#84637,#84638));
#18722=EDGE_LOOP('',(#84639,#84640,#84641,#84642));
#18723=EDGE_LOOP('',(#84643,#84644,#84645,#84646,#84647));
#18724=EDGE_LOOP('',(#84648,#84649,#84650,#84651));
#18725=EDGE_LOOP('',(#84652,#84653,#84654,#84655));
#18726=EDGE_LOOP('',(#84656,#84657,#84658,#84659));
#18727=EDGE_LOOP('',(#84660,#84661,#84662,#84663));
#18728=EDGE_LOOP('',(#84664,#84665,#84666,#84667,#84668));
#18729=EDGE_LOOP('',(#84669,#84670,#84671,#84672));
#18730=EDGE_LOOP('',(#84673,#84674,#84675,#84676));
#18731=EDGE_LOOP('',(#84677,#84678,#84679,#84680));
#18732=EDGE_LOOP('',(#84681,#84682,#84683,#84684));
#18733=EDGE_LOOP('',(#84685,#84686,#84687,#84688));
#18734=EDGE_LOOP('',(#84689,#84690,#84691,#84692));
#18735=EDGE_LOOP('',(#84693,#84694,#84695,#84696));
#18736=EDGE_LOOP('',(#84697,#84698,#84699,#84700));
#18737=EDGE_LOOP('',(#84701,#84702,#84703,#84704));
#18738=EDGE_LOOP('',(#84705,#84706,#84707,#84708));
#18739=EDGE_LOOP('',(#84709,#84710,#84711,#84712,#84713));
#18740=EDGE_LOOP('',(#84714,#84715,#84716,#84717));
#18741=EDGE_LOOP('',(#84718,#84719,#84720,#84721));
#18742=EDGE_LOOP('',(#84722,#84723,#84724,#84725));
#18743=EDGE_LOOP('',(#84726,#84727,#84728,#84729));
#18744=EDGE_LOOP('',(#84730,#84731,#84732,#84733));
#18745=EDGE_LOOP('',(#84734,#84735,#84736,#84737));
#18746=EDGE_LOOP('',(#84738,#84739,#84740,#84741));
#18747=EDGE_LOOP('',(#84742,#84743,#84744,#84745));
#18748=EDGE_LOOP('',(#84746,#84747,#84748,#84749,#84750));
#18749=EDGE_LOOP('',(#84751,#84752,#84753,#84754));
#18750=EDGE_LOOP('',(#84755,#84756,#84757,#84758));
#18751=EDGE_LOOP('',(#84759,#84760,#84761,#84762,#84763));
#18752=EDGE_LOOP('',(#84764,#84765,#84766,#84767));
#18753=EDGE_LOOP('',(#84768,#84769,#84770,#84771));
#18754=EDGE_LOOP('',(#84772,#84773,#84774,#84775));
#18755=EDGE_LOOP('',(#84776,#84777,#84778,#84779));
#18756=EDGE_LOOP('',(#84780,#84781,#84782,#84783,#84784));
#18757=EDGE_LOOP('',(#84785,#84786,#84787,#84788));
#18758=EDGE_LOOP('',(#84789,#84790,#84791,#84792));
#18759=EDGE_LOOP('',(#84793,#84794,#84795,#84796));
#18760=EDGE_LOOP('',(#84797,#84798,#84799,#84800));
#18761=EDGE_LOOP('',(#84801,#84802,#84803,#84804));
#18762=EDGE_LOOP('',(#84805,#84806,#84807,#84808));
#18763=EDGE_LOOP('',(#84809,#84810,#84811,#84812));
#18764=EDGE_LOOP('',(#84813,#84814,#84815,#84816));
#18765=EDGE_LOOP('',(#84817,#84818,#84819,#84820));
#18766=EDGE_LOOP('',(#84821,#84822,#84823,#84824));
#18767=EDGE_LOOP('',(#84825,#84826,#84827,#84828,#84829));
#18768=EDGE_LOOP('',(#84830,#84831,#84832,#84833));
#18769=EDGE_LOOP('',(#84834,#84835,#84836,#84837));
#18770=EDGE_LOOP('',(#84838,#84839,#84840,#84841));
#18771=EDGE_LOOP('',(#84842,#84843,#84844,#84845));
#18772=EDGE_LOOP('',(#84846,#84847,#84848,#84849));
#18773=EDGE_LOOP('',(#84850,#84851,#84852,#84853));
#18774=EDGE_LOOP('',(#84854,#84855,#84856,#84857));
#18775=EDGE_LOOP('',(#84858,#84859,#84860,#84861));
#18776=EDGE_LOOP('',(#84862,#84863,#84864,#84865,#84866));
#18777=EDGE_LOOP('',(#84867,#84868,#84869,#84870));
#18778=EDGE_LOOP('',(#84871,#84872,#84873,#84874));
#18779=EDGE_LOOP('',(#84875,#84876,#84877,#84878,#84879));
#18780=EDGE_LOOP('',(#84880,#84881,#84882,#84883));
#18781=EDGE_LOOP('',(#84884,#84885,#84886,#84887));
#18782=EDGE_LOOP('',(#84888,#84889,#84890,#84891));
#18783=EDGE_LOOP('',(#84892,#84893,#84894,#84895));
#18784=EDGE_LOOP('',(#84896,#84897,#84898,#84899,#84900));
#18785=EDGE_LOOP('',(#84901,#84902,#84903,#84904));
#18786=EDGE_LOOP('',(#84905,#84906,#84907,#84908));
#18787=EDGE_LOOP('',(#84909,#84910,#84911,#84912));
#18788=EDGE_LOOP('',(#84913,#84914,#84915,#84916));
#18789=EDGE_LOOP('',(#84917,#84918,#84919,#84920));
#18790=EDGE_LOOP('',(#84921,#84922,#84923,#84924));
#18791=EDGE_LOOP('',(#84925,#84926,#84927,#84928));
#18792=EDGE_LOOP('',(#84929,#84930,#84931,#84932));
#18793=EDGE_LOOP('',(#84933,#84934,#84935,#84936));
#18794=EDGE_LOOP('',(#84937,#84938,#84939,#84940));
#18795=EDGE_LOOP('',(#84941,#84942,#84943,#84944,#84945));
#18796=EDGE_LOOP('',(#84946,#84947,#84948,#84949));
#18797=EDGE_LOOP('',(#84950,#84951,#84952,#84953));
#18798=EDGE_LOOP('',(#84954,#84955,#84956,#84957));
#18799=EDGE_LOOP('',(#84958,#84959,#84960,#84961));
#18800=EDGE_LOOP('',(#84962,#84963,#84964,#84965));
#18801=EDGE_LOOP('',(#84966,#84967,#84968,#84969));
#18802=EDGE_LOOP('',(#84970,#84971,#84972,#84973));
#18803=EDGE_LOOP('',(#84974,#84975,#84976,#84977));
#18804=EDGE_LOOP('',(#84978,#84979,#84980,#84981,#84982));
#18805=EDGE_LOOP('',(#84983,#84984,#84985,#84986));
#18806=EDGE_LOOP('',(#84987,#84988,#84989,#84990));
#18807=EDGE_LOOP('',(#84991,#84992,#84993,#84994,#84995));
#18808=EDGE_LOOP('',(#84996,#84997,#84998,#84999));
#18809=EDGE_LOOP('',(#85000,#85001,#85002,#85003));
#18810=EDGE_LOOP('',(#85004,#85005,#85006,#85007));
#18811=EDGE_LOOP('',(#85008,#85009,#85010,#85011));
#18812=EDGE_LOOP('',(#85012,#85013,#85014,#85015,#85016));
#18813=EDGE_LOOP('',(#85017,#85018,#85019,#85020));
#18814=EDGE_LOOP('',(#85021,#85022,#85023,#85024));
#18815=EDGE_LOOP('',(#85025,#85026,#85027,#85028));
#18816=EDGE_LOOP('',(#85029,#85030,#85031,#85032));
#18817=EDGE_LOOP('',(#85033,#85034,#85035,#85036));
#18818=EDGE_LOOP('',(#85037,#85038,#85039,#85040));
#18819=EDGE_LOOP('',(#85041,#85042,#85043,#85044));
#18820=EDGE_LOOP('',(#85045,#85046,#85047,#85048));
#18821=EDGE_LOOP('',(#85049,#85050,#85051,#85052));
#18822=EDGE_LOOP('',(#85053,#85054,#85055,#85056));
#18823=EDGE_LOOP('',(#85057,#85058,#85059,#85060,#85061));
#18824=EDGE_LOOP('',(#85062,#85063,#85064,#85065));
#18825=EDGE_LOOP('',(#85066,#85067,#85068,#85069));
#18826=EDGE_LOOP('',(#85070,#85071,#85072,#85073));
#18827=EDGE_LOOP('',(#85074,#85075,#85076,#85077));
#18828=EDGE_LOOP('',(#85078,#85079,#85080,#85081));
#18829=EDGE_LOOP('',(#85082,#85083,#85084,#85085));
#18830=EDGE_LOOP('',(#85086,#85087,#85088,#85089));
#18831=EDGE_LOOP('',(#85090,#85091,#85092,#85093));
#18832=EDGE_LOOP('',(#85094,#85095,#85096,#85097,#85098));
#18833=EDGE_LOOP('',(#85099,#85100,#85101,#85102));
#18834=EDGE_LOOP('',(#85103,#85104,#85105,#85106));
#18835=EDGE_LOOP('',(#85107,#85108,#85109,#85110,#85111));
#18836=EDGE_LOOP('',(#85112,#85113,#85114,#85115));
#18837=EDGE_LOOP('',(#85116,#85117,#85118,#85119));
#18838=EDGE_LOOP('',(#85120,#85121,#85122,#85123));
#18839=EDGE_LOOP('',(#85124,#85125,#85126,#85127));
#18840=EDGE_LOOP('',(#85128,#85129,#85130,#85131,#85132));
#18841=EDGE_LOOP('',(#85133,#85134,#85135,#85136));
#18842=EDGE_LOOP('',(#85137,#85138,#85139,#85140));
#18843=EDGE_LOOP('',(#85141,#85142,#85143,#85144));
#18844=EDGE_LOOP('',(#85145,#85146,#85147,#85148));
#18845=EDGE_LOOP('',(#85149,#85150,#85151,#85152));
#18846=EDGE_LOOP('',(#85153,#85154,#85155,#85156));
#18847=EDGE_LOOP('',(#85157,#85158,#85159,#85160));
#18848=EDGE_LOOP('',(#85161,#85162,#85163,#85164));
#18849=EDGE_LOOP('',(#85165,#85166,#85167,#85168));
#18850=EDGE_LOOP('',(#85169,#85170,#85171,#85172));
#18851=EDGE_LOOP('',(#85173,#85174,#85175,#85176,#85177));
#18852=EDGE_LOOP('',(#85178,#85179,#85180,#85181));
#18853=EDGE_LOOP('',(#85182,#85183,#85184,#85185));
#18854=EDGE_LOOP('',(#85186,#85187,#85188,#85189));
#18855=EDGE_LOOP('',(#85190,#85191,#85192,#85193));
#18856=EDGE_LOOP('',(#85194,#85195,#85196,#85197));
#18857=EDGE_LOOP('',(#85198,#85199,#85200,#85201));
#18858=EDGE_LOOP('',(#85202,#85203,#85204,#85205));
#18859=EDGE_LOOP('',(#85206,#85207,#85208,#85209));
#18860=EDGE_LOOP('',(#85210,#85211,#85212,#85213,#85214));
#18861=EDGE_LOOP('',(#85215,#85216,#85217,#85218));
#18862=EDGE_LOOP('',(#85219,#85220,#85221,#85222));
#18863=EDGE_LOOP('',(#85223,#85224,#85225,#85226,#85227));
#18864=EDGE_LOOP('',(#85228,#85229,#85230,#85231));
#18865=EDGE_LOOP('',(#85232,#85233,#85234,#85235));
#18866=EDGE_LOOP('',(#85236,#85237,#85238,#85239));
#18867=EDGE_LOOP('',(#85240,#85241,#85242,#85243));
#18868=EDGE_LOOP('',(#85244,#85245,#85246,#85247,#85248));
#18869=EDGE_LOOP('',(#85249,#85250,#85251,#85252));
#18870=EDGE_LOOP('',(#85253,#85254,#85255,#85256));
#18871=EDGE_LOOP('',(#85257,#85258,#85259,#85260));
#18872=EDGE_LOOP('',(#85261,#85262,#85263,#85264));
#18873=EDGE_LOOP('',(#85265,#85266,#85267,#85268));
#18874=EDGE_LOOP('',(#85269,#85270,#85271,#85272));
#18875=EDGE_LOOP('',(#85273,#85274,#85275,#85276));
#18876=EDGE_LOOP('',(#85277,#85278,#85279,#85280));
#18877=EDGE_LOOP('',(#85281,#85282,#85283,#85284));
#18878=EDGE_LOOP('',(#85285,#85286,#85287,#85288));
#18879=EDGE_LOOP('',(#85289,#85290,#85291,#85292,#85293));
#18880=EDGE_LOOP('',(#85294,#85295,#85296,#85297));
#18881=EDGE_LOOP('',(#85298,#85299,#85300,#85301));
#18882=EDGE_LOOP('',(#85302,#85303,#85304,#85305));
#18883=EDGE_LOOP('',(#85306,#85307,#85308,#85309));
#18884=EDGE_LOOP('',(#85310,#85311,#85312,#85313));
#18885=EDGE_LOOP('',(#85314,#85315,#85316,#85317));
#18886=EDGE_LOOP('',(#85318,#85319,#85320,#85321));
#18887=EDGE_LOOP('',(#85322,#85323,#85324,#85325));
#18888=EDGE_LOOP('',(#85326,#85327,#85328,#85329,#85330));
#18889=EDGE_LOOP('',(#85331,#85332,#85333,#85334));
#18890=EDGE_LOOP('',(#85335,#85336,#85337,#85338));
#18891=EDGE_LOOP('',(#85339,#85340,#85341,#85342,#85343));
#18892=EDGE_LOOP('',(#85344,#85345,#85346,#85347));
#18893=EDGE_LOOP('',(#85348,#85349,#85350,#85351));
#18894=EDGE_LOOP('',(#85352,#85353,#85354,#85355));
#18895=EDGE_LOOP('',(#85356,#85357,#85358,#85359));
#18896=EDGE_LOOP('',(#85360,#85361,#85362,#85363,#85364));
#18897=EDGE_LOOP('',(#85365,#85366,#85367,#85368));
#18898=EDGE_LOOP('',(#85369,#85370,#85371,#85372));
#18899=EDGE_LOOP('',(#85373,#85374,#85375,#85376));
#18900=EDGE_LOOP('',(#85377,#85378,#85379,#85380));
#18901=EDGE_LOOP('',(#85381,#85382,#85383,#85384));
#18902=EDGE_LOOP('',(#85385,#85386,#85387,#85388));
#18903=EDGE_LOOP('',(#85389,#85390,#85391,#85392));
#18904=EDGE_LOOP('',(#85393,#85394,#85395,#85396));
#18905=EDGE_LOOP('',(#85397,#85398,#85399,#85400));
#18906=EDGE_LOOP('',(#85401,#85402,#85403,#85404));
#18907=EDGE_LOOP('',(#85405,#85406,#85407,#85408,#85409));
#18908=EDGE_LOOP('',(#85410,#85411,#85412,#85413));
#18909=EDGE_LOOP('',(#85414,#85415,#85416,#85417));
#18910=EDGE_LOOP('',(#85418,#85419,#85420,#85421));
#18911=EDGE_LOOP('',(#85422,#85423,#85424,#85425));
#18912=EDGE_LOOP('',(#85426,#85427,#85428,#85429));
#18913=EDGE_LOOP('',(#85430,#85431,#85432,#85433));
#18914=EDGE_LOOP('',(#85434,#85435,#85436,#85437));
#18915=EDGE_LOOP('',(#85438,#85439,#85440,#85441));
#18916=EDGE_LOOP('',(#85442,#85443,#85444,#85445,#85446));
#18917=EDGE_LOOP('',(#85447,#85448,#85449,#85450));
#18918=EDGE_LOOP('',(#85451,#85452,#85453,#85454));
#18919=EDGE_LOOP('',(#85455,#85456,#85457,#85458,#85459));
#18920=EDGE_LOOP('',(#85460,#85461,#85462,#85463));
#18921=EDGE_LOOP('',(#85464,#85465,#85466,#85467));
#18922=EDGE_LOOP('',(#85468,#85469,#85470,#85471));
#18923=EDGE_LOOP('',(#85472,#85473,#85474,#85475));
#18924=EDGE_LOOP('',(#85476,#85477,#85478,#85479,#85480));
#18925=EDGE_LOOP('',(#85481,#85482,#85483,#85484));
#18926=EDGE_LOOP('',(#85485,#85486,#85487,#85488));
#18927=EDGE_LOOP('',(#85489,#85490,#85491,#85492));
#18928=EDGE_LOOP('',(#85493,#85494,#85495,#85496));
#18929=EDGE_LOOP('',(#85497,#85498,#85499,#85500));
#18930=EDGE_LOOP('',(#85501,#85502,#85503,#85504));
#18931=EDGE_LOOP('',(#85505,#85506,#85507,#85508));
#18932=EDGE_LOOP('',(#85509,#85510,#85511,#85512));
#18933=EDGE_LOOP('',(#85513,#85514,#85515,#85516));
#18934=EDGE_LOOP('',(#85517,#85518,#85519,#85520));
#18935=EDGE_LOOP('',(#85521,#85522,#85523,#85524,#85525));
#18936=EDGE_LOOP('',(#85526,#85527,#85528,#85529));
#18937=EDGE_LOOP('',(#85530,#85531,#85532,#85533));
#18938=EDGE_LOOP('',(#85534,#85535,#85536,#85537));
#18939=EDGE_LOOP('',(#85538,#85539,#85540,#85541));
#18940=EDGE_LOOP('',(#85542,#85543,#85544,#85545));
#18941=EDGE_LOOP('',(#85546,#85547,#85548,#85549));
#18942=EDGE_LOOP('',(#85550,#85551,#85552,#85553));
#18943=EDGE_LOOP('',(#85554,#85555,#85556,#85557));
#18944=EDGE_LOOP('',(#85558,#85559,#85560,#85561,#85562));
#18945=EDGE_LOOP('',(#85563,#85564,#85565,#85566));
#18946=EDGE_LOOP('',(#85567,#85568,#85569,#85570));
#18947=EDGE_LOOP('',(#85571,#85572,#85573,#85574,#85575));
#18948=EDGE_LOOP('',(#85576,#85577,#85578,#85579));
#18949=EDGE_LOOP('',(#85580,#85581,#85582,#85583));
#18950=EDGE_LOOP('',(#85584,#85585,#85586,#85587));
#18951=EDGE_LOOP('',(#85588,#85589,#85590,#85591));
#18952=EDGE_LOOP('',(#85592,#85593,#85594,#85595,#85596));
#18953=EDGE_LOOP('',(#85597,#85598,#85599,#85600));
#18954=EDGE_LOOP('',(#85601,#85602,#85603,#85604));
#18955=EDGE_LOOP('',(#85605,#85606,#85607,#85608));
#18956=EDGE_LOOP('',(#85609,#85610,#85611,#85612));
#18957=EDGE_LOOP('',(#85613,#85614,#85615,#85616));
#18958=EDGE_LOOP('',(#85617,#85618,#85619,#85620));
#18959=EDGE_LOOP('',(#85621,#85622,#85623,#85624));
#18960=EDGE_LOOP('',(#85625,#85626,#85627,#85628));
#18961=EDGE_LOOP('',(#85629,#85630,#85631,#85632));
#18962=EDGE_LOOP('',(#85633,#85634,#85635,#85636));
#18963=EDGE_LOOP('',(#85637,#85638,#85639,#85640,#85641));
#18964=EDGE_LOOP('',(#85642,#85643,#85644,#85645));
#18965=EDGE_LOOP('',(#85646,#85647,#85648,#85649));
#18966=EDGE_LOOP('',(#85650,#85651,#85652,#85653));
#18967=EDGE_LOOP('',(#85654,#85655,#85656,#85657));
#18968=EDGE_LOOP('',(#85658,#85659,#85660,#85661));
#18969=EDGE_LOOP('',(#85662,#85663,#85664,#85665));
#18970=EDGE_LOOP('',(#85666,#85667,#85668,#85669));
#18971=EDGE_LOOP('',(#85670,#85671,#85672,#85673));
#18972=EDGE_LOOP('',(#85674,#85675,#85676,#85677,#85678));
#18973=EDGE_LOOP('',(#85679,#85680,#85681,#85682));
#18974=EDGE_LOOP('',(#85683,#85684,#85685,#85686));
#18975=EDGE_LOOP('',(#85687,#85688,#85689,#85690,#85691));
#18976=EDGE_LOOP('',(#85692,#85693,#85694,#85695));
#18977=EDGE_LOOP('',(#85696,#85697,#85698,#85699));
#18978=EDGE_LOOP('',(#85700,#85701,#85702,#85703));
#18979=EDGE_LOOP('',(#85704,#85705,#85706,#85707));
#18980=EDGE_LOOP('',(#85708,#85709,#85710,#85711,#85712));
#18981=EDGE_LOOP('',(#85713,#85714,#85715,#85716));
#18982=EDGE_LOOP('',(#85717,#85718,#85719,#85720));
#18983=EDGE_LOOP('',(#85721,#85722,#85723,#85724));
#18984=EDGE_LOOP('',(#85725,#85726,#85727,#85728));
#18985=EDGE_LOOP('',(#85729,#85730,#85731,#85732));
#18986=EDGE_LOOP('',(#85733,#85734,#85735,#85736));
#18987=EDGE_LOOP('',(#85737,#85738,#85739,#85740));
#18988=EDGE_LOOP('',(#85741,#85742,#85743,#85744));
#18989=EDGE_LOOP('',(#85745,#85746,#85747,#85748));
#18990=EDGE_LOOP('',(#85749,#85750,#85751,#85752));
#18991=EDGE_LOOP('',(#85753,#85754,#85755,#85756,#85757));
#18992=EDGE_LOOP('',(#85758,#85759,#85760,#85761));
#18993=EDGE_LOOP('',(#85762,#85763,#85764,#85765));
#18994=EDGE_LOOP('',(#85766,#85767,#85768,#85769));
#18995=EDGE_LOOP('',(#85770,#85771,#85772,#85773));
#18996=EDGE_LOOP('',(#85774,#85775,#85776,#85777));
#18997=EDGE_LOOP('',(#85778,#85779,#85780,#85781));
#18998=EDGE_LOOP('',(#85782,#85783,#85784,#85785));
#18999=EDGE_LOOP('',(#85786,#85787,#85788,#85789));
#19000=EDGE_LOOP('',(#85790,#85791,#85792,#85793,#85794));
#19001=EDGE_LOOP('',(#85795,#85796,#85797,#85798));
#19002=EDGE_LOOP('',(#85799,#85800,#85801,#85802));
#19003=EDGE_LOOP('',(#85803,#85804,#85805,#85806,#85807));
#19004=EDGE_LOOP('',(#85808,#85809,#85810,#85811));
#19005=EDGE_LOOP('',(#85812,#85813,#85814,#85815,#85816));
#19006=EDGE_LOOP('',(#85817,#85818,#85819,#85820));
#19007=EDGE_LOOP('',(#85821));
#19008=EDGE_LOOP('',(#85822));
#19009=EDGE_LOOP('',(#85823));
#19010=EDGE_LOOP('',(#85824));
#19011=EDGE_LOOP('',(#85825));
#19012=EDGE_LOOP('',(#85826));
#19013=EDGE_LOOP('',(#85827,#85828,#85829,#85830));
#19014=EDGE_LOOP('',(#85831,#85832,#85833,#85834));
#19015=EDGE_LOOP('',(#85835,#85836,#85837,#85838));
#19016=EDGE_LOOP('',(#85839,#85840,#85841,#85842));
#19017=EDGE_LOOP('',(#85843));
#19018=EDGE_LOOP('',(#85844));
#19019=EDGE_LOOP('',(#85845));
#19020=EDGE_LOOP('',(#85846));
#19021=EDGE_LOOP('',(#85847,#85848,#85849,#85850));
#19022=EDGE_LOOP('',(#85851,#85852,#85853,#85854));
#19023=EDGE_LOOP('',(#85855,#85856,#85857,#85858));
#19024=EDGE_LOOP('',(#85859,#85860,#85861,#85862));
#19025=EDGE_LOOP('',(#85863,#85864,#85865,#85866));
#19026=EDGE_LOOP('',(#85867,#85868,#85869,#85870));
#19027=EDGE_LOOP('',(#85871,#85872,#85873,#85874));
#19028=EDGE_LOOP('',(#85875,#85876,#85877,#85878));
#19029=EDGE_LOOP('',(#85879,#85880,#85881,#85882));
#19030=EDGE_LOOP('',(#85883,#85884,#85885,#85886,#85887,#85888));
#19031=EDGE_LOOP('',(#85889,#85890,#85891,#85892,#85893,#85894));
#19032=EDGE_LOOP('',(#85895,#85896,#85897,#85898));
#19033=EDGE_LOOP('',(#85899,#85900,#85901,#85902));
#19034=EDGE_LOOP('',(#85903,#85904,#85905,#85906));
#19035=EDGE_LOOP('',(#85907,#85908,#85909,#85910));
#19036=EDGE_LOOP('',(#85911,#85912,#85913,#85914));
#19037=EDGE_LOOP('',(#85915,#85916,#85917,#85918));
#19038=EDGE_LOOP('',(#85919,#85920,#85921,#85922));
#19039=EDGE_LOOP('',(#85923,#85924,#85925,#85926,#85927,#85928,#85929,#85930,
#85931,#85932,#85933,#85934,#85935,#85936,#85937,#85938,#85939,#85940,#85941,
#85942,#85943,#85944,#85945,#85946,#85947,#85948,#85949,#85950));
#19040=EDGE_LOOP('',(#85951,#85952,#85953,#85954,#85955,#85956,#85957,#85958,
#85959,#85960));
#19041=EDGE_LOOP('',(#85961,#85962,#85963,#85964,#85965,#85966,#85967,#85968,
#85969,#85970));
#19042=EDGE_LOOP('',(#85971,#85972,#85973,#85974));
#19043=EDGE_LOOP('',(#85975,#85976,#85977,#85978));
#19044=EDGE_LOOP('',(#85979,#85980,#85981,#85982));
#19045=EDGE_LOOP('',(#85983,#85984,#85985,#85986,#85987,#85988,#85989,#85990,
#85991,#85992));
#19046=EDGE_LOOP('',(#85993,#85994,#85995,#85996,#85997,#85998,#85999,#86000,
#86001,#86002));
#19047=EDGE_LOOP('',(#86003,#86004,#86005,#86006,#86007,#86008));
#19048=EDGE_LOOP('',(#86009,#86010,#86011,#86012));
#19049=EDGE_LOOP('',(#86013,#86014,#86015,#86016));
#19050=EDGE_LOOP('',(#86017,#86018,#86019,#86020));
#19051=EDGE_LOOP('',(#86021,#86022,#86023,#86024));
#19052=EDGE_LOOP('',(#86025,#86026,#86027,#86028));
#19053=EDGE_LOOP('',(#86029,#86030,#86031,#86032));
#19054=EDGE_LOOP('',(#86033,#86034,#86035,#86036));
#19055=EDGE_LOOP('',(#86037,#86038,#86039,#86040));
#19056=EDGE_LOOP('',(#86041,#86042,#86043,#86044,#86045,#86046));
#19057=EDGE_LOOP('',(#86047));
#19058=EDGE_LOOP('',(#86048,#86049,#86050,#86051,#86052,#86053,#86054,#86055));
#19059=EDGE_LOOP('',(#86056,#86057,#86058,#86059,#86060,#86061,#86062,#86063));
#19060=EDGE_LOOP('',(#86064,#86065,#86066,#86067));
#19061=EDGE_LOOP('',(#86068,#86069,#86070,#86071,#86072,#86073));
#19062=EDGE_LOOP('',(#86074,#86075,#86076,#86077));
#19063=EDGE_LOOP('',(#86078,#86079,#86080,#86081,#86082,#86083,#86084));
#19064=EDGE_LOOP('',(#86085,#86086,#86087,#86088,#86089,#86090,#86091));
#19065=EDGE_LOOP('',(#86092,#86093,#86094,#86095));
#19066=EDGE_LOOP('',(#86096,#86097,#86098,#86099));
#19067=EDGE_LOOP('',(#86100));
#19068=EDGE_LOOP('',(#86101,#86102,#86103,#86104));
#19069=EDGE_LOOP('',(#86105,#86106,#86107,#86108));
#19070=EDGE_LOOP('',(#86109));
#19071=EDGE_LOOP('',(#86110,#86111,#86112,#86113));
#19072=EDGE_LOOP('',(#86114,#86115,#86116,#86117));
#19073=EDGE_LOOP('',(#86118));
#19074=EDGE_LOOP('',(#86119,#86120,#86121,#86122));
#19075=EDGE_LOOP('',(#86123));
#19076=EDGE_LOOP('',(#86124,#86125,#86126,#86127,#86128,#86129));
#19077=EDGE_LOOP('',(#86130,#86131,#86132,#86133,#86134,#86135));
#19078=EDGE_LOOP('',(#86136,#86137,#86138,#86139,#86140,#86141));
#19079=EDGE_LOOP('',(#86142,#86143,#86144,#86145,#86146,#86147,#86148,#86149));
#19080=EDGE_LOOP('',(#86150,#86151,#86152,#86153,#86154,#86155));
#19081=EDGE_LOOP('',(#86156,#86157,#86158,#86159,#86160,#86161));
#19082=EDGE_LOOP('',(#86162,#86163,#86164,#86165,#86166,#86167,#86168,#86169));
#19083=EDGE_LOOP('',(#86170,#86171,#86172,#86173,#86174,#86175));
#19084=EDGE_LOOP('',(#86176,#86177,#86178,#86179,#86180,#86181));
#19085=EDGE_LOOP('',(#86182,#86183,#86184,#86185,#86186,#86187,#86188,#86189));
#19086=EDGE_LOOP('',(#86190,#86191,#86192,#86193,#86194));
#19087=EDGE_LOOP('',(#86195,#86196,#86197,#86198,#86199,#86200,#86201,#86202));
#19088=EDGE_LOOP('',(#86203));
#19089=EDGE_LOOP('',(#86204));
#19090=EDGE_LOOP('',(#86205));
#19091=EDGE_LOOP('',(#86206));
#19092=EDGE_LOOP('',(#86207));
#19093=EDGE_LOOP('',(#86208));
#19094=EDGE_LOOP('',(#86209));
#19095=EDGE_LOOP('',(#86210,#86211,#86212,#86213,#86214,#86215,#86216,#86217));
#19096=EDGE_LOOP('',(#86218,#86219,#86220,#86221,#86222,#86223,#86224,#86225));
#19097=EDGE_LOOP('',(#86226,#86227,#86228,#86229));
#19098=EDGE_LOOP('',(#86230,#86231,#86232,#86233));
#19099=EDGE_LOOP('',(#86234,#86235,#86236,#86237));
#19100=EDGE_LOOP('',(#86238,#86239,#86240,#86241));
#19101=EDGE_LOOP('',(#86242,#86243,#86244,#86245,#86246));
#19102=EDGE_LOOP('',(#86247,#86248,#86249,#86250));
#19103=EDGE_LOOP('',(#86251,#86252,#86253,#86254,#86255));
#19104=EDGE_LOOP('',(#86256,#86257,#86258,#86259));
#19105=EDGE_LOOP('',(#86260,#86261,#86262,#86263,#86264));
#19106=EDGE_LOOP('',(#86265,#86266,#86267,#86268));
#19107=EDGE_LOOP('',(#86269,#86270,#86271,#86272,#86273,#86274));
#19108=EDGE_LOOP('',(#86275,#86276,#86277,#86278));
#19109=EDGE_LOOP('',(#86279,#86280,#86281,#86282,#86283));
#19110=EDGE_LOOP('',(#86284,#86285,#86286,#86287));
#19111=EDGE_LOOP('',(#86288,#86289,#86290,#86291,#86292));
#19112=EDGE_LOOP('',(#86293,#86294,#86295,#86296));
#19113=EDGE_LOOP('',(#86297,#86298,#86299,#86300));
#19114=EDGE_LOOP('',(#86301,#86302,#86303,#86304));
#19115=EDGE_LOOP('',(#86305,#86306,#86307,#86308));
#19116=EDGE_LOOP('',(#86309,#86310,#86311,#86312));
#19117=EDGE_LOOP('',(#86313,#86314,#86315,#86316));
#19118=EDGE_LOOP('',(#86317,#86318,#86319,#86320));
#19119=EDGE_LOOP('',(#86321,#86322,#86323,#86324));
#19120=EDGE_LOOP('',(#86325,#86326,#86327));
#19121=EDGE_LOOP('',(#86328,#86329,#86330,#86331));
#19122=EDGE_LOOP('',(#86332,#86333,#86334,#86335));
#19123=EDGE_LOOP('',(#86336,#86337,#86338,#86339));
#19124=EDGE_LOOP('',(#86340,#86341,#86342));
#19125=EDGE_LOOP('',(#86343,#86344,#86345,#86346));
#19126=EDGE_LOOP('',(#86347,#86348,#86349,#86350));
#19127=EDGE_LOOP('',(#86351,#86352,#86353));
#19128=EDGE_LOOP('',(#86354,#86355,#86356,#86357));
#19129=EDGE_LOOP('',(#86358,#86359,#86360,#86361));
#19130=EDGE_LOOP('',(#86362,#86363,#86364,#86365));
#19131=EDGE_LOOP('',(#86366,#86367,#86368));
#19132=EDGE_LOOP('',(#86369,#86370,#86371,#86372));
#19133=EDGE_LOOP('',(#86373,#86374,#86375,#86376));
#19134=EDGE_LOOP('',(#86377,#86378,#86379,#86380));
#19135=EDGE_LOOP('',(#86381,#86382,#86383));
#19136=EDGE_LOOP('',(#86384,#86385,#86386,#86387));
#19137=EDGE_LOOP('',(#86388,#86389,#86390,#86391));
#19138=EDGE_LOOP('',(#86392,#86393,#86394,#86395));
#19139=EDGE_LOOP('',(#86396,#86397,#86398));
#19140=EDGE_LOOP('',(#86399,#86400,#86401,#86402));
#19141=EDGE_LOOP('',(#86403,#86404,#86405,#86406));
#19142=EDGE_LOOP('',(#86407,#86408,#86409,#86410));
#19143=EDGE_LOOP('',(#86411,#86412,#86413,#86414));
#19144=EDGE_LOOP('',(#86415,#86416,#86417,#86418));
#19145=EDGE_LOOP('',(#86419,#86420,#86421,#86422));
#19146=EDGE_LOOP('',(#86423,#86424,#86425,#86426));
#19147=EDGE_LOOP('',(#86427,#86428,#86429,#86430));
#19148=EDGE_LOOP('',(#86431,#86432,#86433,#86434));
#19149=EDGE_LOOP('',(#86435,#86436,#86437,#86438));
#19150=EDGE_LOOP('',(#86439,#86440,#86441,#86442));
#19151=EDGE_LOOP('',(#86443,#86444,#86445,#86446));
#19152=EDGE_LOOP('',(#86447,#86448,#86449,#86450));
#19153=EDGE_LOOP('',(#86451,#86452,#86453,#86454,#86455,#86456));
#19154=EDGE_LOOP('',(#86457,#86458,#86459,#86460));
#19155=EDGE_LOOP('',(#86461,#86462,#86463,#86464,#86465,#86466));
#19156=EDGE_LOOP('',(#86467,#86468,#86469,#86470,#86471,#86472));
#19157=EDGE_LOOP('',(#86473,#86474,#86475,#86476));
#19158=EDGE_LOOP('',(#86477,#86478,#86479,#86480,#86481,#86482));
#19159=EDGE_LOOP('',(#86483,#86484,#86485,#86486,#86487,#86488));
#19160=EDGE_LOOP('',(#86489,#86490,#86491,#86492));
#19161=EDGE_LOOP('',(#86493,#86494,#86495,#86496,#86497,#86498));
#19162=EDGE_LOOP('',(#86499,#86500,#86501,#86502,#86503,#86504));
#19163=EDGE_LOOP('',(#86505,#86506,#86507,#86508));
#19164=EDGE_LOOP('',(#86509,#86510,#86511,#86512,#86513,#86514));
#19165=EDGE_LOOP('',(#86515,#86516,#86517,#86518));
#19166=EDGE_LOOP('',(#86519,#86520,#86521,#86522));
#19167=EDGE_LOOP('',(#86523,#86524,#86525,#86526,#86527));
#19168=EDGE_LOOP('',(#86528,#86529,#86530,#86531));
#19169=EDGE_LOOP('',(#86532,#86533,#86534,#86535));
#19170=EDGE_LOOP('',(#86536,#86537,#86538,#86539,#86540));
#19171=EDGE_LOOP('',(#86541,#86542,#86543,#86544,#86545));
#19172=EDGE_LOOP('',(#86546,#86547,#86548));
#19173=EDGE_LOOP('',(#86549,#86550,#86551,#86552,#86553));
#19174=EDGE_LOOP('',(#86554,#86555,#86556));
#19175=EDGE_LOOP('',(#86557,#86558,#86559,#86560));
#19176=EDGE_LOOP('',(#86561,#86562,#86563));
#19177=EDGE_LOOP('',(#86564,#86565,#86566));
#19178=EDGE_LOOP('',(#86567,#86568,#86569,#86570));
#19179=EDGE_LOOP('',(#86571,#86572,#86573,#86574));
#19180=EDGE_LOOP('',(#86575,#86576,#86577));
#19181=EDGE_LOOP('',(#86578,#86579,#86580,#86581));
#19182=EDGE_LOOP('',(#86582,#86583,#86584,#86585));
#19183=EDGE_LOOP('',(#86586,#86587,#86588));
#19184=EDGE_LOOP('',(#86589,#86590,#86591,#86592));
#19185=EDGE_LOOP('',(#86593,#86594,#86595,#86596));
#19186=EDGE_LOOP('',(#86597,#86598,#86599));
#19187=EDGE_LOOP('',(#86600,#86601,#86602,#86603,#86604));
#19188=EDGE_LOOP('',(#86605,#86606,#86607,#86608));
#19189=EDGE_LOOP('',(#86609,#86610,#86611));
#19190=EDGE_LOOP('',(#86612,#86613,#86614,#86615,#86616));
#19191=EDGE_LOOP('',(#86617,#86618,#86619,#86620));
#19192=EDGE_LOOP('',(#86621,#86622,#86623));
#19193=EDGE_LOOP('',(#86624,#86625,#86626,#86627));
#19194=EDGE_LOOP('',(#86628,#86629,#86630,#86631));
#19195=EDGE_LOOP('',(#86632,#86633,#86634));
#19196=EDGE_LOOP('',(#86635,#86636,#86637));
#19197=EDGE_LOOP('',(#86638,#86639,#86640,#86641));
#19198=EDGE_LOOP('',(#86642,#86643,#86644,#86645));
#19199=EDGE_LOOP('',(#86646,#86647,#86648,#86649));
#19200=EDGE_LOOP('',(#86650,#86651,#86652,#86653));
#19201=EDGE_LOOP('',(#86654,#86655,#86656));
#19202=EDGE_LOOP('',(#86657,#86658,#86659,#86660));
#19203=EDGE_LOOP('',(#86661,#86662,#86663,#86664));
#19204=EDGE_LOOP('',(#86665,#86666,#86667,#86668));
#19205=EDGE_LOOP('',(#86669,#86670,#86671,#86672));
#19206=EDGE_LOOP('',(#86673,#86674,#86675,#86676));
#19207=EDGE_LOOP('',(#86677,#86678));
#19208=EDGE_LOOP('',(#86679,#86680,#86681,#86682,#86683));
#19209=EDGE_LOOP('',(#86684,#86685,#86686,#86687,#86688));
#19210=EDGE_LOOP('',(#86689,#86690,#86691,#86692,#86693,#86694));
#19211=EDGE_LOOP('',(#86695,#86696,#86697,#86698));
#19212=EDGE_LOOP('',(#86699,#86700,#86701,#86702,#86703,#86704,#86705));
#19213=EDGE_LOOP('',(#86706,#86707,#86708,#86709,#86710,#86711));
#19214=EDGE_LOOP('',(#86712,#86713,#86714));
#19215=EDGE_LOOP('',(#86715));
#19216=EDGE_LOOP('',(#86716));
#19217=EDGE_LOOP('',(#86717,#86718,#86719,#86720,#86721,#86722));
#19218=EDGE_LOOP('',(#86723,#86724,#86725,#86726,#86727));
#19219=EDGE_LOOP('',(#86728,#86729,#86730,#86731,#86732));
#19220=EDGE_LOOP('',(#86733,#86734,#86735,#86736,#86737));
#19221=EDGE_LOOP('',(#86738,#86739,#86740,#86741,#86742));
#19222=EDGE_LOOP('',(#86743));
#19223=EDGE_LOOP('',(#86744,#86745,#86746,#86747,#86748));
#19224=EDGE_LOOP('',(#86749,#86750));
#19225=EDGE_LOOP('',(#86751));
#19226=EDGE_LOOP('',(#86752));
#19227=EDGE_LOOP('',(#86753));
#19228=EDGE_LOOP('',(#86754));
#19229=EDGE_LOOP('',(#86755,#86756,#86757,#86758));
#19230=EDGE_LOOP('',(#86759,#86760,#86761,#86762,#86763));
#19231=EDGE_LOOP('',(#86764,#86765,#86766,#86767,#86768));
#19232=EDGE_LOOP('',(#86769,#86770,#86771,#86772));
#19233=EDGE_LOOP('',(#86773,#86774,#86775,#86776));
#19234=EDGE_LOOP('',(#86777,#86778,#86779,#86780));
#19235=EDGE_LOOP('',(#86781,#86782,#86783,#86784));
#19236=EDGE_LOOP('',(#86785,#86786,#86787,#86788));
#19237=EDGE_LOOP('',(#86789,#86790,#86791,#86792,#86793));
#19238=EDGE_LOOP('',(#86794,#86795,#86796,#86797,#86798));
#19239=EDGE_LOOP('',(#86799,#86800,#86801,#86802));
#19240=EDGE_LOOP('',(#86803));
#19241=EDGE_LOOP('',(#86804));
#19242=EDGE_LOOP('',(#86805));
#19243=EDGE_LOOP('',(#86806));
#19244=EDGE_LOOP('',(#86807));
#19245=EDGE_LOOP('',(#86808));
#19246=EDGE_LOOP('',(#86809));
#19247=EDGE_LOOP('',(#86810));
#19248=EDGE_LOOP('',(#86811));
#19249=EDGE_LOOP('',(#86812));
#19250=EDGE_LOOP('',(#86813,#86814,#86815,#86816));
#19251=EDGE_LOOP('',(#86817,#86818,#86819,#86820));
#19252=EDGE_LOOP('',(#86821,#86822,#86823,#86824));
#19253=EDGE_LOOP('',(#86825,#86826,#86827,#86828));
#19254=EDGE_LOOP('',(#86829,#86830,#86831,#86832));
#19255=EDGE_LOOP('',(#86833,#86834,#86835,#86836));
#19256=EDGE_LOOP('',(#86837,#86838,#86839));
#19257=EDGE_LOOP('',(#86840,#86841,#86842,#86843,#86844));
#19258=EDGE_LOOP('',(#86845,#86846,#86847,#86848));
#19259=EDGE_LOOP('',(#86849,#86850,#86851,#86852));
#19260=EDGE_LOOP('',(#86853,#86854,#86855,#86856));
#19261=EDGE_LOOP('',(#86857,#86858,#86859,#86860));
#19262=EDGE_LOOP('',(#86861,#86862,#86863,#86864));
#19263=EDGE_LOOP('',(#86865,#86866,#86867,#86868,#86869));
#19264=EDGE_LOOP('',(#86870,#86871,#86872,#86873,#86874,#86875,#86876,#86877));
#19265=EDGE_LOOP('',(#86878,#86879,#86880,#86881,#86882,#86883,#86884,#86885,
#86886));
#19266=EDGE_LOOP('',(#86887,#86888,#86889,#86890));
#19267=EDGE_LOOP('',(#86891));
#19268=EDGE_LOOP('',(#86892));
#19269=EDGE_LOOP('',(#86893,#86894,#86895,#86896,#86897,#86898));
#19270=EDGE_LOOP('',(#86899,#86900));
#19271=EDGE_LOOP('',(#86901,#86902));
#19272=EDGE_LOOP('',(#86903,#86904));
#19273=EDGE_LOOP('',(#86905,#86906));
#19274=EDGE_LOOP('',(#86907,#86908));
#19275=EDGE_LOOP('',(#86909,#86910));
#19276=EDGE_LOOP('',(#86911,#86912,#86913,#86914,#86915,#86916));
#19277=EDGE_LOOP('',(#86917,#86918,#86919,#86920));
#19278=EDGE_LOOP('',(#86921,#86922,#86923,#86924));
#19279=EDGE_LOOP('',(#86925,#86926,#86927,#86928));
#19280=EDGE_LOOP('',(#86929,#86930,#86931,#86932));
#19281=EDGE_LOOP('',(#86933,#86934,#86935,#86936));
#19282=EDGE_LOOP('',(#86937,#86938,#86939,#86940));
#19283=EDGE_LOOP('',(#86941,#86942,#86943,#86944,#86945,#86946,#86947,#86948,
#86949,#86950,#86951,#86952,#86953,#86954,#86955,#86956,#86957));
#19284=EDGE_LOOP('',(#86958,#86959,#86960,#86961));
#19285=EDGE_LOOP('',(#86962,#86963,#86964,#86965,#86966,#86967,#86968,#86969,
#86970,#86971,#86972,#86973,#86974,#86975,#86976,#86977,#86978));
#19286=EDGE_LOOP('',(#86979,#86980,#86981,#86982));
#19287=EDGE_LOOP('',(#86983,#86984,#86985,#86986));
#19288=EDGE_LOOP('',(#86987,#86988,#86989,#86990));
#19289=EDGE_LOOP('',(#86991,#86992,#86993,#86994));
#19290=EDGE_LOOP('',(#86995,#86996,#86997,#86998));
#19291=EDGE_LOOP('',(#86999,#87000,#87001,#87002));
#19292=EDGE_LOOP('',(#87003,#87004,#87005));
#19293=EDGE_LOOP('',(#87006,#87007,#87008,#87009,#87010));
#19294=EDGE_LOOP('',(#87011,#87012,#87013,#87014));
#19295=EDGE_LOOP('',(#87015,#87016,#87017,#87018));
#19296=EDGE_LOOP('',(#87019,#87020,#87021,#87022));
#19297=EDGE_LOOP('',(#87023,#87024,#87025,#87026));
#19298=EDGE_LOOP('',(#87027,#87028,#87029,#87030));
#19299=EDGE_LOOP('',(#87031,#87032,#87033,#87034,#87035));
#19300=EDGE_LOOP('',(#87036,#87037,#87038,#87039,#87040,#87041,#87042,#87043));
#19301=EDGE_LOOP('',(#87044,#87045,#87046,#87047,#87048,#87049,#87050,#87051,
#87052));
#19302=EDGE_LOOP('',(#87053,#87054,#87055,#87056));
#19303=EDGE_LOOP('',(#87057));
#19304=EDGE_LOOP('',(#87058));
#19305=EDGE_LOOP('',(#87059,#87060,#87061,#87062,#87063,#87064));
#19306=EDGE_LOOP('',(#87065,#87066));
#19307=EDGE_LOOP('',(#87067,#87068));
#19308=EDGE_LOOP('',(#87069,#87070));
#19309=EDGE_LOOP('',(#87071,#87072));
#19310=EDGE_LOOP('',(#87073,#87074));
#19311=EDGE_LOOP('',(#87075,#87076));
#19312=EDGE_LOOP('',(#87077,#87078,#87079,#87080,#87081,#87082));
#19313=EDGE_LOOP('',(#87083,#87084,#87085,#87086));
#19314=EDGE_LOOP('',(#87087,#87088,#87089,#87090));
#19315=EDGE_LOOP('',(#87091,#87092,#87093,#87094));
#19316=EDGE_LOOP('',(#87095,#87096,#87097,#87098));
#19317=EDGE_LOOP('',(#87099,#87100,#87101,#87102));
#19318=EDGE_LOOP('',(#87103,#87104,#87105,#87106));
#19319=EDGE_LOOP('',(#87107,#87108,#87109,#87110,#87111,#87112,#87113,#87114,
#87115,#87116,#87117,#87118,#87119,#87120,#87121,#87122,#87123));
#19320=EDGE_LOOP('',(#87124,#87125,#87126,#87127));
#19321=EDGE_LOOP('',(#87128,#87129,#87130,#87131,#87132,#87133,#87134,#87135,
#87136,#87137,#87138,#87139,#87140,#87141,#87142,#87143,#87144));
#19322=EDGE_LOOP('',(#87145,#87146,#87147,#87148));
#19323=EDGE_LOOP('',(#87149,#87150,#87151,#87152,#87153));
#19324=EDGE_LOOP('',(#87154,#87155,#87156,#87157));
#19325=EDGE_LOOP('',(#87158,#87159,#87160,#87161,#87162));
#19326=EDGE_LOOP('',(#87163,#87164,#87165,#87166,#87167,#87168,#87169,#87170,
#87171));
#19327=EDGE_LOOP('',(#87172,#87173));
#19328=EDGE_LOOP('',(#87174,#87175,#87176,#87177,#87178));
#19329=EDGE_LOOP('',(#87179,#87180,#87181,#87182,#87183,#87184));
#19330=EDGE_LOOP('',(#87185,#87186,#87187,#87188,#87189,#87190,#87191,#87192,
#87193));
#19331=EDGE_LOOP('',(#87194));
#19332=EDGE_LOOP('',(#87195));
#19333=EDGE_LOOP('',(#87196));
#19334=EDGE_LOOP('',(#87197));
#19335=EDGE_LOOP('',(#87198));
#19336=EDGE_LOOP('',(#87199,#87200,#87201,#87202));
#19337=EDGE_LOOP('',(#87203,#87204,#87205,#87206));
#19338=EDGE_LOOP('',(#87207,#87208,#87209,#87210,#87211));
#19339=EDGE_LOOP('',(#87212,#87213,#87214,#87215,#87216));
#19340=EDGE_LOOP('',(#87217,#87218,#87219,#87220));
#19341=EDGE_LOOP('',(#87221,#87222,#87223,#87224));
#19342=EDGE_LOOP('',(#87225,#87226,#87227,#87228));
#19343=EDGE_LOOP('',(#87229,#87230,#87231,#87232));
#19344=EDGE_LOOP('',(#87233,#87234,#87235,#87236));
#19345=EDGE_LOOP('',(#87237,#87238,#87239,#87240));
#19346=EDGE_LOOP('',(#87241,#87242,#87243,#87244));
#19347=EDGE_LOOP('',(#87245,#87246,#87247,#87248));
#19348=EDGE_LOOP('',(#87249,#87250,#87251,#87252));
#19349=EDGE_LOOP('',(#87253,#87254,#87255,#87256));
#19350=EDGE_LOOP('',(#87257,#87258,#87259,#87260));
#19351=EDGE_LOOP('',(#87261,#87262,#87263,#87264));
#19352=EDGE_LOOP('',(#87265,#87266,#87267,#87268));
#19353=EDGE_LOOP('',(#87269,#87270,#87271,#87272));
#19354=EDGE_LOOP('',(#87273,#87274,#87275,#87276));
#19355=EDGE_LOOP('',(#87277,#87278,#87279,#87280));
#19356=EDGE_LOOP('',(#87281,#87282,#87283,#87284));
#19357=EDGE_LOOP('',(#87285,#87286,#87287,#87288));
#19358=EDGE_LOOP('',(#87289,#87290,#87291,#87292));
#19359=EDGE_LOOP('',(#87293,#87294,#87295,#87296,#87297,#87298,#87299,#87300));
#19360=EDGE_LOOP('',(#87301));
#19361=EDGE_LOOP('',(#87302));
#19362=EDGE_LOOP('',(#87303));
#19363=EDGE_LOOP('',(#87304));
#19364=EDGE_LOOP('',(#87305));
#19365=EDGE_LOOP('',(#87306));
#19366=EDGE_LOOP('',(#87307));
#19367=EDGE_LOOP('',(#87308));
#19368=EDGE_LOOP('',(#87309));
#19369=EDGE_LOOP('',(#87310));
#19370=EDGE_LOOP('',(#87311));
#19371=EDGE_LOOP('',(#87312));
#19372=EDGE_LOOP('',(#87313));
#19373=EDGE_LOOP('',(#87314,#87315,#87316,#87317,#87318,#87319,#87320,#87321));
#19374=EDGE_LOOP('',(#87322,#87323,#87324,#87325,#87326,#87327,#87328,#87329));
#19375=EDGE_LOOP('',(#87330,#87331,#87332,#87333));
#19376=EDGE_LOOP('',(#87334,#87335,#87336,#87337));
#19377=EDGE_LOOP('',(#87338,#87339,#87340,#87341));
#19378=EDGE_LOOP('',(#87342,#87343,#87344,#87345));
#19379=EDGE_LOOP('',(#87346,#87347,#87348,#87349));
#19380=EDGE_LOOP('',(#87350,#87351,#87352,#87353));
#19381=EDGE_LOOP('',(#87354,#87355,#87356,#87357));
#19382=EDGE_LOOP('',(#87358,#87359,#87360,#87361));
#19383=EDGE_LOOP('',(#87362,#87363,#87364,#87365));
#19384=EDGE_LOOP('',(#87366,#87367,#87368,#87369));
#19385=EDGE_LOOP('',(#87370,#87371,#87372,#87373));
#19386=EDGE_LOOP('',(#87374,#87375,#87376,#87377));
#19387=EDGE_LOOP('',(#87378,#87379,#87380,#87381));
#19388=EDGE_LOOP('',(#87382,#87383,#87384,#87385));
#19389=EDGE_LOOP('',(#87386,#87387,#87388,#87389));
#19390=EDGE_LOOP('',(#87390,#87391,#87392,#87393));
#19391=EDGE_LOOP('',(#87394,#87395,#87396,#87397,#87398,#87399,#87400,#87401));
#19392=EDGE_LOOP('',(#87402));
#19393=EDGE_LOOP('',(#87403));
#19394=EDGE_LOOP('',(#87404));
#19395=EDGE_LOOP('',(#87405));
#19396=EDGE_LOOP('',(#87406));
#19397=EDGE_LOOP('',(#87407,#87408,#87409,#87410));
#19398=EDGE_LOOP('',(#87411));
#19399=EDGE_LOOP('',(#87412,#87413,#87414,#87415,#87416,#87417,#87418,#87419));
#19400=EDGE_LOOP('',(#87420));
#19401=EDGE_LOOP('',(#87421));
#19402=EDGE_LOOP('',(#87422));
#19403=EDGE_LOOP('',(#87423));
#19404=EDGE_LOOP('',(#87424));
#19405=EDGE_LOOP('',(#87425));
#19406=EDGE_LOOP('',(#87426,#87427,#87428,#87429));
#19407=EDGE_LOOP('',(#87430,#87431,#87432,#87433));
#19408=EDGE_LOOP('',(#87434,#87435,#87436,#87437));
#19409=EDGE_LOOP('',(#87438,#87439,#87440,#87441,#87442,#87443,#87444,#87445));
#19410=EDGE_LOOP('',(#87446));
#19411=EDGE_LOOP('',(#87447,#87448,#87449,#87450));
#19412=EDGE_LOOP('',(#87451,#87452,#87453,#87454));
#19413=EDGE_LOOP('',(#87455,#87456,#87457,#87458));
#20078=LINE('',#167167,#25305);
#20079=LINE('',#167179,#25306);
#20080=LINE('',#167194,#25307);
#20081=LINE('',#167227,#25308);
#20082=LINE('',#167242,#25309);
#20083=LINE('',#167254,#25310);
#20084=LINE('',#167448,#25311);
#20085=LINE('',#167450,#25312);
#20086=LINE('',#167451,#25313);
#20087=LINE('',#167453,#25314);
#20088=LINE('',#167454,#25315);
#20089=LINE('',#167456,#25316);
#20090=LINE('',#167457,#25317);
#20091=LINE('',#167459,#25318);
#20092=LINE('',#167460,#25319);
#20093=LINE('',#167462,#25320);
#20094=LINE('',#167472,#25321);
#20095=LINE('',#167478,#25322);
#20096=LINE('',#167486,#25323);
#20097=LINE('',#167492,#25324);
#20098=LINE('',#167500,#25325);
#20099=LINE('',#167506,#25326);
#20100=LINE('',#167514,#25327);
#20101=LINE('',#167520,#25328);
#20102=LINE('',#167543,#25329);
#20103=LINE('',#167546,#25330);
#20104=LINE('',#167569,#25331);
#20105=LINE('',#167572,#25332);
#20106=LINE('',#167580,#25333);
#20107=LINE('',#167586,#25334);
#20108=LINE('',#167660,#25335);
#20109=LINE('',#167663,#25336);
#20110=LINE('',#167713,#25337);
#20111=LINE('',#167717,#25338);
#20112=LINE('',#167806,#25339);
#20113=LINE('',#167810,#25340);
#20114=LINE('',#167899,#25341);
#20115=LINE('',#167903,#25342);
#20116=LINE('',#167992,#25343);
#20117=LINE('',#167996,#25344);
#20118=LINE('',#168085,#25345);
#20119=LINE('',#168089,#25346);
#20120=LINE('',#168178,#25347);
#20121=LINE('',#168182,#25348);
#20122=LINE('',#168271,#25349);
#20123=LINE('',#168275,#25350);
#20124=LINE('',#168364,#25351);
#20125=LINE('',#168368,#25352);
#20126=LINE('',#168457,#25353);
#20127=LINE('',#168461,#25354);
#20128=LINE('',#168550,#25355);
#20129=LINE('',#168554,#25356);
#20130=LINE('',#168643,#25357);
#20131=LINE('',#168647,#25358);
#20132=LINE('',#168736,#25359);
#20133=LINE('',#168740,#25360);
#20134=LINE('',#168829,#25361);
#20135=LINE('',#168833,#25362);
#20136=LINE('',#168922,#25363);
#20137=LINE('',#168926,#25364);
#20138=LINE('',#169015,#25365);
#20139=LINE('',#169019,#25366);
#20140=LINE('',#169108,#25367);
#20141=LINE('',#169112,#25368);
#20142=LINE('',#169201,#25369);
#20143=LINE('',#169205,#25370);
#20144=LINE('',#169294,#25371);
#20145=LINE('',#169298,#25372);
#20146=LINE('',#169387,#25373);
#20147=LINE('',#169391,#25374);
#20148=LINE('',#169480,#25375);
#20149=LINE('',#169484,#25376);
#20150=LINE('',#169573,#25377);
#20151=LINE('',#169577,#25378);
#20152=LINE('',#169666,#25379);
#20153=LINE('',#169670,#25380);
#20154=LINE('',#169759,#25381);
#20155=LINE('',#169763,#25382);
#20156=LINE('',#169852,#25383);
#20157=LINE('',#169856,#25384);
#20158=LINE('',#169945,#25385);
#20159=LINE('',#169949,#25386);
#20160=LINE('',#170038,#25387);
#20161=LINE('',#170042,#25388);
#20162=LINE('',#170131,#25389);
#20163=LINE('',#170135,#25390);
#20164=LINE('',#170224,#25391);
#20165=LINE('',#170228,#25392);
#20166=LINE('',#170317,#25393);
#20167=LINE('',#170321,#25394);
#20168=LINE('',#170410,#25395);
#20169=LINE('',#170414,#25396);
#20170=LINE('',#170455,#25397);
#20171=LINE('',#170501,#25398);
#20172=LINE('',#170505,#25399);
#20173=LINE('',#170594,#25400);
#20174=LINE('',#170598,#25401);
#20175=LINE('',#170687,#25402);
#20176=LINE('',#170691,#25403);
#20177=LINE('',#170780,#25404);
#20178=LINE('',#170784,#25405);
#20179=LINE('',#170873,#25406);
#20180=LINE('',#170877,#25407);
#20181=LINE('',#170966,#25408);
#20182=LINE('',#170970,#25409);
#20183=LINE('',#171059,#25410);
#20184=LINE('',#171063,#25411);
#20185=LINE('',#171152,#25412);
#20186=LINE('',#171156,#25413);
#20187=LINE('',#171245,#25414);
#20188=LINE('',#171249,#25415);
#20189=LINE('',#171338,#25416);
#20190=LINE('',#171342,#25417);
#20191=LINE('',#171431,#25418);
#20192=LINE('',#171435,#25419);
#20193=LINE('',#171524,#25420);
#20194=LINE('',#171528,#25421);
#20195=LINE('',#171617,#25422);
#20196=LINE('',#171621,#25423);
#20197=LINE('',#171710,#25424);
#20198=LINE('',#171714,#25425);
#20199=LINE('',#171803,#25426);
#20200=LINE('',#171807,#25427);
#20201=LINE('',#171893,#25428);
#20202=LINE('',#171897,#25429);
#20203=LINE('',#171986,#25430);
#20204=LINE('',#171990,#25431);
#20205=LINE('',#172079,#25432);
#20206=LINE('',#172083,#25433);
#20207=LINE('',#172172,#25434);
#20208=LINE('',#172176,#25435);
#20209=LINE('',#172265,#25436);
#20210=LINE('',#172269,#25437);
#20211=LINE('',#172358,#25438);
#20212=LINE('',#172362,#25439);
#20213=LINE('',#172451,#25440);
#20214=LINE('',#172455,#25441);
#20215=LINE('',#172544,#25442);
#20216=LINE('',#172548,#25443);
#20217=LINE('',#172637,#25444);
#20218=LINE('',#172641,#25445);
#20219=LINE('',#172730,#25446);
#20220=LINE('',#172734,#25447);
#20221=LINE('',#172823,#25448);
#20222=LINE('',#172827,#25449);
#20223=LINE('',#172916,#25450);
#20224=LINE('',#172920,#25451);
#20225=LINE('',#173009,#25452);
#20226=LINE('',#173013,#25453);
#20227=LINE('',#173102,#25454);
#20228=LINE('',#173106,#25455);
#20229=LINE('',#173195,#25456);
#20230=LINE('',#173199,#25457);
#20231=LINE('',#173280,#25458);
#20232=LINE('',#173284,#25459);
#20233=LINE('',#173367,#25460);
#20234=LINE('',#173371,#25461);
#20235=LINE('',#173454,#25462);
#20236=LINE('',#173458,#25463);
#20237=LINE('',#173541,#25464);
#20238=LINE('',#173545,#25465);
#20239=LINE('',#173628,#25466);
#20240=LINE('',#173632,#25467);
#20241=LINE('',#173715,#25468);
#20242=LINE('',#173719,#25469);
#20243=LINE('',#173802,#25470);
#20244=LINE('',#173806,#25471);
#20245=LINE('',#173889,#25472);
#20246=LINE('',#173893,#25473);
#20247=LINE('',#173976,#25474);
#20248=LINE('',#173980,#25475);
#20249=LINE('',#174063,#25476);
#20250=LINE('',#174067,#25477);
#20251=LINE('',#174150,#25478);
#20252=LINE('',#174154,#25479);
#20253=LINE('',#174237,#25480);
#20254=LINE('',#174241,#25481);
#20255=LINE('',#174324,#25482);
#20256=LINE('',#174328,#25483);
#20257=LINE('',#174411,#25484);
#20258=LINE('',#174415,#25485);
#20259=LINE('',#174498,#25486);
#20260=LINE('',#174502,#25487);
#20261=LINE('',#174585,#25488);
#20262=LINE('',#174589,#25489);
#20263=LINE('',#174672,#25490);
#20264=LINE('',#174676,#25491);
#20265=LINE('',#174759,#25492);
#20266=LINE('',#174763,#25493);
#20267=LINE('',#174846,#25494);
#20268=LINE('',#174850,#25495);
#20269=LINE('',#174933,#25496);
#20270=LINE('',#174937,#25497);
#20271=LINE('',#175020,#25498);
#20272=LINE('',#175024,#25499);
#20273=LINE('',#175107,#25500);
#20274=LINE('',#175111,#25501);
#20275=LINE('',#175194,#25502);
#20276=LINE('',#175198,#25503);
#20277=LINE('',#175281,#25504);
#20278=LINE('',#175285,#25505);
#20279=LINE('',#175368,#25506);
#20280=LINE('',#175372,#25507);
#20281=LINE('',#175455,#25508);
#20282=LINE('',#175459,#25509);
#20283=LINE('',#175542,#25510);
#20284=LINE('',#175546,#25511);
#20285=LINE('',#175629,#25512);
#20286=LINE('',#175633,#25513);
#20287=LINE('',#175716,#25514);
#20288=LINE('',#175720,#25515);
#20289=LINE('',#175803,#25516);
#20290=LINE('',#175807,#25517);
#20291=LINE('',#175851,#25518);
#20292=LINE('',#175893,#25519);
#20293=LINE('',#175897,#25520);
#20294=LINE('',#175980,#25521);
#20295=LINE('',#175984,#25522);
#20296=LINE('',#176067,#25523);
#20297=LINE('',#176071,#25524);
#20298=LINE('',#176154,#25525);
#20299=LINE('',#176158,#25526);
#20300=LINE('',#176241,#25527);
#20301=LINE('',#176245,#25528);
#20302=LINE('',#176328,#25529);
#20303=LINE('',#176332,#25530);
#20304=LINE('',#176415,#25531);
#20305=LINE('',#176419,#25532);
#20306=LINE('',#176502,#25533);
#20307=LINE('',#176506,#25534);
#20308=LINE('',#176589,#25535);
#20309=LINE('',#176593,#25536);
#20310=LINE('',#176676,#25537);
#20311=LINE('',#176680,#25538);
#20312=LINE('',#176763,#25539);
#20313=LINE('',#176767,#25540);
#20314=LINE('',#176850,#25541);
#20315=LINE('',#176854,#25542);
#20316=LINE('',#176937,#25543);
#20317=LINE('',#176941,#25544);
#20318=LINE('',#177024,#25545);
#20319=LINE('',#177028,#25546);
#20320=LINE('',#177111,#25547);
#20321=LINE('',#177115,#25548);
#20322=LINE('',#177195,#25549);
#20323=LINE('',#177199,#25550);
#20324=LINE('',#177282,#25551);
#20325=LINE('',#177286,#25552);
#20326=LINE('',#177369,#25553);
#20327=LINE('',#177373,#25554);
#20328=LINE('',#177456,#25555);
#20329=LINE('',#177460,#25556);
#20330=LINE('',#177543,#25557);
#20331=LINE('',#177547,#25558);
#20332=LINE('',#177630,#25559);
#20333=LINE('',#177634,#25560);
#20334=LINE('',#177717,#25561);
#20335=LINE('',#177721,#25562);
#20336=LINE('',#177804,#25563);
#20337=LINE('',#177808,#25564);
#20338=LINE('',#177891,#25565);
#20339=LINE('',#177895,#25566);
#20340=LINE('',#177978,#25567);
#20341=LINE('',#177982,#25568);
#20342=LINE('',#178065,#25569);
#20343=LINE('',#178069,#25570);
#20344=LINE('',#178152,#25571);
#20345=LINE('',#178156,#25572);
#20346=LINE('',#178239,#25573);
#20347=LINE('',#178243,#25574);
#20348=LINE('',#178326,#25575);
#20349=LINE('',#178330,#25576);
#20350=LINE('',#178413,#25577);
#20351=LINE('',#178417,#25578);
#20352=LINE('',#178462,#25579);
#20353=LINE('',#178466,#25580);
#20354=LINE('',#178473,#25581);
#20355=LINE('',#178477,#25582);
#20356=LINE('',#178485,#25583);
#20357=LINE('',#178486,#25584);
#20358=LINE('',#178492,#25585);
#20359=LINE('',#178495,#25586);
#20360=LINE('',#178501,#25587);
#20361=LINE('',#178505,#25588);
#20362=LINE('',#178513,#25589);
#20363=LINE('',#178514,#25590);
#20364=LINE('',#178532,#25591);
#20365=LINE('',#178539,#25592);
#20366=LINE('',#178542,#25593);
#20367=LINE('',#178545,#25594);
#20368=LINE('',#178551,#25595);
#20369=LINE('',#178554,#25596);
#20370=LINE('',#178560,#25597);
#20371=LINE('',#178567,#25598);
#20372=LINE('',#178570,#25599);
#20373=LINE('',#178573,#25600);
#20374=LINE('',#178591,#25601);
#20375=LINE('',#178598,#25602);
#20376=LINE('',#178601,#25603);
#20377=LINE('',#178604,#25604);
#20378=LINE('',#178610,#25605);
#20379=LINE('',#178613,#25606);
#20380=LINE('',#178619,#25607);
#20381=LINE('',#178626,#25608);
#20382=LINE('',#178629,#25609);
#20383=LINE('',#178632,#25610);
#20384=LINE('',#178650,#25611);
#20385=LINE('',#178657,#25612);
#20386=LINE('',#178660,#25613);
#20387=LINE('',#178663,#25614);
#20388=LINE('',#178669,#25615);
#20389=LINE('',#178672,#25616);
#20390=LINE('',#178678,#25617);
#20391=LINE('',#178685,#25618);
#20392=LINE('',#178688,#25619);
#20393=LINE('',#178691,#25620);
#20394=LINE('',#178709,#25621);
#20395=LINE('',#178716,#25622);
#20396=LINE('',#178719,#25623);
#20397=LINE('',#178722,#25624);
#20398=LINE('',#178728,#25625);
#20399=LINE('',#178731,#25626);
#20400=LINE('',#178737,#25627);
#20401=LINE('',#178744,#25628);
#20402=LINE('',#178747,#25629);
#20403=LINE('',#178750,#25630);
#20404=LINE('',#178768,#25631);
#20405=LINE('',#178775,#25632);
#20406=LINE('',#178778,#25633);
#20407=LINE('',#178781,#25634);
#20408=LINE('',#178787,#25635);
#20409=LINE('',#178790,#25636);
#20410=LINE('',#178796,#25637);
#20411=LINE('',#178803,#25638);
#20412=LINE('',#178806,#25639);
#20413=LINE('',#178809,#25640);
#20414=LINE('',#178827,#25641);
#20415=LINE('',#178834,#25642);
#20416=LINE('',#178837,#25643);
#20417=LINE('',#178840,#25644);
#20418=LINE('',#178846,#25645);
#20419=LINE('',#178849,#25646);
#20420=LINE('',#178855,#25647);
#20421=LINE('',#178862,#25648);
#20422=LINE('',#178865,#25649);
#20423=LINE('',#178868,#25650);
#20424=LINE('',#178886,#25651);
#20425=LINE('',#178893,#25652);
#20426=LINE('',#178896,#25653);
#20427=LINE('',#178899,#25654);
#20428=LINE('',#178905,#25655);
#20429=LINE('',#178908,#25656);
#20430=LINE('',#178914,#25657);
#20431=LINE('',#178921,#25658);
#20432=LINE('',#178924,#25659);
#20433=LINE('',#178927,#25660);
#20434=LINE('',#178945,#25661);
#20435=LINE('',#178952,#25662);
#20436=LINE('',#178955,#25663);
#20437=LINE('',#178958,#25664);
#20438=LINE('',#178964,#25665);
#20439=LINE('',#178967,#25666);
#20440=LINE('',#178973,#25667);
#20441=LINE('',#178980,#25668);
#20442=LINE('',#178983,#25669);
#20443=LINE('',#178986,#25670);
#20444=LINE('',#179004,#25671);
#20445=LINE('',#179011,#25672);
#20446=LINE('',#179014,#25673);
#20447=LINE('',#179017,#25674);
#20448=LINE('',#179023,#25675);
#20449=LINE('',#179026,#25676);
#20450=LINE('',#179032,#25677);
#20451=LINE('',#179039,#25678);
#20452=LINE('',#179042,#25679);
#20453=LINE('',#179045,#25680);
#20454=LINE('',#179063,#25681);
#20455=LINE('',#179070,#25682);
#20456=LINE('',#179073,#25683);
#20457=LINE('',#179076,#25684);
#20458=LINE('',#179082,#25685);
#20459=LINE('',#179085,#25686);
#20460=LINE('',#179091,#25687);
#20461=LINE('',#179098,#25688);
#20462=LINE('',#179101,#25689);
#20463=LINE('',#179104,#25690);
#20464=LINE('',#179122,#25691);
#20465=LINE('',#179129,#25692);
#20466=LINE('',#179132,#25693);
#20467=LINE('',#179135,#25694);
#20468=LINE('',#179141,#25695);
#20469=LINE('',#179144,#25696);
#20470=LINE('',#179150,#25697);
#20471=LINE('',#179157,#25698);
#20472=LINE('',#179160,#25699);
#20473=LINE('',#179163,#25700);
#20474=LINE('',#179181,#25701);
#20475=LINE('',#179188,#25702);
#20476=LINE('',#179191,#25703);
#20477=LINE('',#179194,#25704);
#20478=LINE('',#179200,#25705);
#20479=LINE('',#179203,#25706);
#20480=LINE('',#179209,#25707);
#20481=LINE('',#179216,#25708);
#20482=LINE('',#179219,#25709);
#20483=LINE('',#179222,#25710);
#20484=LINE('',#179240,#25711);
#20485=LINE('',#179247,#25712);
#20486=LINE('',#179250,#25713);
#20487=LINE('',#179253,#25714);
#20488=LINE('',#179259,#25715);
#20489=LINE('',#179262,#25716);
#20490=LINE('',#179268,#25717);
#20491=LINE('',#179275,#25718);
#20492=LINE('',#179278,#25719);
#20493=LINE('',#179281,#25720);
#20494=LINE('',#179299,#25721);
#20495=LINE('',#179306,#25722);
#20496=LINE('',#179309,#25723);
#20497=LINE('',#179312,#25724);
#20498=LINE('',#179318,#25725);
#20499=LINE('',#179321,#25726);
#20500=LINE('',#179327,#25727);
#20501=LINE('',#179334,#25728);
#20502=LINE('',#179337,#25729);
#20503=LINE('',#179340,#25730);
#20504=LINE('',#179358,#25731);
#20505=LINE('',#179365,#25732);
#20506=LINE('',#179368,#25733);
#20507=LINE('',#179371,#25734);
#20508=LINE('',#179377,#25735);
#20509=LINE('',#179380,#25736);
#20510=LINE('',#179386,#25737);
#20511=LINE('',#179393,#25738);
#20512=LINE('',#179396,#25739);
#20513=LINE('',#179399,#25740);
#20514=LINE('',#179417,#25741);
#20515=LINE('',#179424,#25742);
#20516=LINE('',#179427,#25743);
#20517=LINE('',#179430,#25744);
#20518=LINE('',#179436,#25745);
#20519=LINE('',#179439,#25746);
#20520=LINE('',#179445,#25747);
#20521=LINE('',#179452,#25748);
#20522=LINE('',#179455,#25749);
#20523=LINE('',#179458,#25750);
#20524=LINE('',#179476,#25751);
#20525=LINE('',#179483,#25752);
#20526=LINE('',#179486,#25753);
#20527=LINE('',#179489,#25754);
#20528=LINE('',#179495,#25755);
#20529=LINE('',#179498,#25756);
#20530=LINE('',#179504,#25757);
#20531=LINE('',#179511,#25758);
#20532=LINE('',#179514,#25759);
#20533=LINE('',#179517,#25760);
#20534=LINE('',#179535,#25761);
#20535=LINE('',#179542,#25762);
#20536=LINE('',#179545,#25763);
#20537=LINE('',#179548,#25764);
#20538=LINE('',#179554,#25765);
#20539=LINE('',#179557,#25766);
#20540=LINE('',#179563,#25767);
#20541=LINE('',#179570,#25768);
#20542=LINE('',#179573,#25769);
#20543=LINE('',#179576,#25770);
#20544=LINE('',#179594,#25771);
#20545=LINE('',#179601,#25772);
#20546=LINE('',#179604,#25773);
#20547=LINE('',#179607,#25774);
#20548=LINE('',#179613,#25775);
#20549=LINE('',#179616,#25776);
#20550=LINE('',#179622,#25777);
#20551=LINE('',#179629,#25778);
#20552=LINE('',#179632,#25779);
#20553=LINE('',#179635,#25780);
#20554=LINE('',#179653,#25781);
#20555=LINE('',#179660,#25782);
#20556=LINE('',#179663,#25783);
#20557=LINE('',#179666,#25784);
#20558=LINE('',#179672,#25785);
#20559=LINE('',#179675,#25786);
#20560=LINE('',#179681,#25787);
#20561=LINE('',#179688,#25788);
#20562=LINE('',#179691,#25789);
#20563=LINE('',#179694,#25790);
#20564=LINE('',#179712,#25791);
#20565=LINE('',#179719,#25792);
#20566=LINE('',#179722,#25793);
#20567=LINE('',#179725,#25794);
#20568=LINE('',#179731,#25795);
#20569=LINE('',#179734,#25796);
#20570=LINE('',#179740,#25797);
#20571=LINE('',#179747,#25798);
#20572=LINE('',#179750,#25799);
#20573=LINE('',#179753,#25800);
#20574=LINE('',#179771,#25801);
#20575=LINE('',#179778,#25802);
#20576=LINE('',#179781,#25803);
#20577=LINE('',#179784,#25804);
#20578=LINE('',#179790,#25805);
#20579=LINE('',#179793,#25806);
#20580=LINE('',#179799,#25807);
#20581=LINE('',#179806,#25808);
#20582=LINE('',#179809,#25809);
#20583=LINE('',#179812,#25810);
#20584=LINE('',#179830,#25811);
#20585=LINE('',#179837,#25812);
#20586=LINE('',#179840,#25813);
#20587=LINE('',#179843,#25814);
#20588=LINE('',#179849,#25815);
#20589=LINE('',#179852,#25816);
#20590=LINE('',#179858,#25817);
#20591=LINE('',#179865,#25818);
#20592=LINE('',#179868,#25819);
#20593=LINE('',#179871,#25820);
#20594=LINE('',#179889,#25821);
#20595=LINE('',#179896,#25822);
#20596=LINE('',#179899,#25823);
#20597=LINE('',#179902,#25824);
#20598=LINE('',#179908,#25825);
#20599=LINE('',#179911,#25826);
#20600=LINE('',#179917,#25827);
#20601=LINE('',#179924,#25828);
#20602=LINE('',#179927,#25829);
#20603=LINE('',#179930,#25830);
#20604=LINE('',#179948,#25831);
#20605=LINE('',#179955,#25832);
#20606=LINE('',#179958,#25833);
#20607=LINE('',#179961,#25834);
#20608=LINE('',#179967,#25835);
#20609=LINE('',#179970,#25836);
#20610=LINE('',#179976,#25837);
#20611=LINE('',#179983,#25838);
#20612=LINE('',#179986,#25839);
#20613=LINE('',#179989,#25840);
#20614=LINE('',#180007,#25841);
#20615=LINE('',#180014,#25842);
#20616=LINE('',#180017,#25843);
#20617=LINE('',#180020,#25844);
#20618=LINE('',#180026,#25845);
#20619=LINE('',#180029,#25846);
#20620=LINE('',#180035,#25847);
#20621=LINE('',#180042,#25848);
#20622=LINE('',#180045,#25849);
#20623=LINE('',#180048,#25850);
#20624=LINE('',#180066,#25851);
#20625=LINE('',#180073,#25852);
#20626=LINE('',#180076,#25853);
#20627=LINE('',#180079,#25854);
#20628=LINE('',#180085,#25855);
#20629=LINE('',#180088,#25856);
#20630=LINE('',#180094,#25857);
#20631=LINE('',#180101,#25858);
#20632=LINE('',#180104,#25859);
#20633=LINE('',#180107,#25860);
#20634=LINE('',#180125,#25861);
#20635=LINE('',#180132,#25862);
#20636=LINE('',#180135,#25863);
#20637=LINE('',#180138,#25864);
#20638=LINE('',#180144,#25865);
#20639=LINE('',#180147,#25866);
#20640=LINE('',#180153,#25867);
#20641=LINE('',#180160,#25868);
#20642=LINE('',#180163,#25869);
#20643=LINE('',#180166,#25870);
#20644=LINE('',#180184,#25871);
#20645=LINE('',#180191,#25872);
#20646=LINE('',#180194,#25873);
#20647=LINE('',#180197,#25874);
#20648=LINE('',#180203,#25875);
#20649=LINE('',#180206,#25876);
#20650=LINE('',#180212,#25877);
#20651=LINE('',#180219,#25878);
#20652=LINE('',#180222,#25879);
#20653=LINE('',#180225,#25880);
#20654=LINE('',#180243,#25881);
#20655=LINE('',#180250,#25882);
#20656=LINE('',#180253,#25883);
#20657=LINE('',#180256,#25884);
#20658=LINE('',#180262,#25885);
#20659=LINE('',#180265,#25886);
#20660=LINE('',#180271,#25887);
#20661=LINE('',#180278,#25888);
#20662=LINE('',#180281,#25889);
#20663=LINE('',#180284,#25890);
#20664=LINE('',#180302,#25891);
#20665=LINE('',#180309,#25892);
#20666=LINE('',#180312,#25893);
#20667=LINE('',#180315,#25894);
#20668=LINE('',#180321,#25895);
#20669=LINE('',#180324,#25896);
#20670=LINE('',#180330,#25897);
#20671=LINE('',#180337,#25898);
#20672=LINE('',#180340,#25899);
#20673=LINE('',#180343,#25900);
#20674=LINE('',#180361,#25901);
#20675=LINE('',#180368,#25902);
#20676=LINE('',#180371,#25903);
#20677=LINE('',#180374,#25904);
#20678=LINE('',#180380,#25905);
#20679=LINE('',#180383,#25906);
#20680=LINE('',#180389,#25907);
#20681=LINE('',#180396,#25908);
#20682=LINE('',#180399,#25909);
#20683=LINE('',#180402,#25910);
#20684=LINE('',#180420,#25911);
#20685=LINE('',#180427,#25912);
#20686=LINE('',#180430,#25913);
#20687=LINE('',#180433,#25914);
#20688=LINE('',#180439,#25915);
#20689=LINE('',#180442,#25916);
#20690=LINE('',#180448,#25917);
#20691=LINE('',#180455,#25918);
#20692=LINE('',#180458,#25919);
#20693=LINE('',#180461,#25920);
#20694=LINE('',#180479,#25921);
#20695=LINE('',#180486,#25922);
#20696=LINE('',#180489,#25923);
#20697=LINE('',#180492,#25924);
#20698=LINE('',#180498,#25925);
#20699=LINE('',#180501,#25926);
#20700=LINE('',#180507,#25927);
#20701=LINE('',#180514,#25928);
#20702=LINE('',#180517,#25929);
#20703=LINE('',#180520,#25930);
#20704=LINE('',#180538,#25931);
#20705=LINE('',#180545,#25932);
#20706=LINE('',#180548,#25933);
#20707=LINE('',#180551,#25934);
#20708=LINE('',#180557,#25935);
#20709=LINE('',#180560,#25936);
#20710=LINE('',#180566,#25937);
#20711=LINE('',#180573,#25938);
#20712=LINE('',#180576,#25939);
#20713=LINE('',#180579,#25940);
#20714=LINE('',#180597,#25941);
#20715=LINE('',#180604,#25942);
#20716=LINE('',#180607,#25943);
#20717=LINE('',#180610,#25944);
#20718=LINE('',#180616,#25945);
#20719=LINE('',#180619,#25946);
#20720=LINE('',#180625,#25947);
#20721=LINE('',#180632,#25948);
#20722=LINE('',#180635,#25949);
#20723=LINE('',#180638,#25950);
#20724=LINE('',#180656,#25951);
#20725=LINE('',#180663,#25952);
#20726=LINE('',#180666,#25953);
#20727=LINE('',#180669,#25954);
#20728=LINE('',#180675,#25955);
#20729=LINE('',#180678,#25956);
#20730=LINE('',#180684,#25957);
#20731=LINE('',#180691,#25958);
#20732=LINE('',#180694,#25959);
#20733=LINE('',#180697,#25960);
#20734=LINE('',#180715,#25961);
#20735=LINE('',#180722,#25962);
#20736=LINE('',#180725,#25963);
#20737=LINE('',#180728,#25964);
#20738=LINE('',#180734,#25965);
#20739=LINE('',#180737,#25966);
#20740=LINE('',#180743,#25967);
#20741=LINE('',#180750,#25968);
#20742=LINE('',#180753,#25969);
#20743=LINE('',#180756,#25970);
#20744=LINE('',#180774,#25971);
#20745=LINE('',#180781,#25972);
#20746=LINE('',#180784,#25973);
#20747=LINE('',#180787,#25974);
#20748=LINE('',#180793,#25975);
#20749=LINE('',#180796,#25976);
#20750=LINE('',#180802,#25977);
#20751=LINE('',#180809,#25978);
#20752=LINE('',#180812,#25979);
#20753=LINE('',#180815,#25980);
#20754=LINE('',#180833,#25981);
#20755=LINE('',#180840,#25982);
#20756=LINE('',#180843,#25983);
#20757=LINE('',#180846,#25984);
#20758=LINE('',#180852,#25985);
#20759=LINE('',#180855,#25986);
#20760=LINE('',#180861,#25987);
#20761=LINE('',#180868,#25988);
#20762=LINE('',#180871,#25989);
#20763=LINE('',#180874,#25990);
#20764=LINE('',#180892,#25991);
#20765=LINE('',#180899,#25992);
#20766=LINE('',#180902,#25993);
#20767=LINE('',#180905,#25994);
#20768=LINE('',#180911,#25995);
#20769=LINE('',#180914,#25996);
#20770=LINE('',#180920,#25997);
#20771=LINE('',#180927,#25998);
#20772=LINE('',#180930,#25999);
#20773=LINE('',#180933,#26000);
#20774=LINE('',#180951,#26001);
#20775=LINE('',#180958,#26002);
#20776=LINE('',#180961,#26003);
#20777=LINE('',#180964,#26004);
#20778=LINE('',#180970,#26005);
#20779=LINE('',#180973,#26006);
#20780=LINE('',#180979,#26007);
#20781=LINE('',#180986,#26008);
#20782=LINE('',#180989,#26009);
#20783=LINE('',#180992,#26010);
#20784=LINE('',#181010,#26011);
#20785=LINE('',#181017,#26012);
#20786=LINE('',#181020,#26013);
#20787=LINE('',#181023,#26014);
#20788=LINE('',#181029,#26015);
#20789=LINE('',#181032,#26016);
#20790=LINE('',#181038,#26017);
#20791=LINE('',#181045,#26018);
#20792=LINE('',#181048,#26019);
#20793=LINE('',#181051,#26020);
#20794=LINE('',#181069,#26021);
#20795=LINE('',#181076,#26022);
#20796=LINE('',#181079,#26023);
#20797=LINE('',#181082,#26024);
#20798=LINE('',#181088,#26025);
#20799=LINE('',#181091,#26026);
#20800=LINE('',#181097,#26027);
#20801=LINE('',#181104,#26028);
#20802=LINE('',#181107,#26029);
#20803=LINE('',#181110,#26030);
#20804=LINE('',#181128,#26031);
#20805=LINE('',#181135,#26032);
#20806=LINE('',#181138,#26033);
#20807=LINE('',#181141,#26034);
#20808=LINE('',#181147,#26035);
#20809=LINE('',#181150,#26036);
#20810=LINE('',#181156,#26037);
#20811=LINE('',#181163,#26038);
#20812=LINE('',#181166,#26039);
#20813=LINE('',#181169,#26040);
#20814=LINE('',#181187,#26041);
#20815=LINE('',#181194,#26042);
#20816=LINE('',#181197,#26043);
#20817=LINE('',#181200,#26044);
#20818=LINE('',#181206,#26045);
#20819=LINE('',#181209,#26046);
#20820=LINE('',#181215,#26047);
#20821=LINE('',#181222,#26048);
#20822=LINE('',#181225,#26049);
#20823=LINE('',#181228,#26050);
#20824=LINE('',#181246,#26051);
#20825=LINE('',#181253,#26052);
#20826=LINE('',#181256,#26053);
#20827=LINE('',#181259,#26054);
#20828=LINE('',#181265,#26055);
#20829=LINE('',#181268,#26056);
#20830=LINE('',#181274,#26057);
#20831=LINE('',#181281,#26058);
#20832=LINE('',#181284,#26059);
#20833=LINE('',#181287,#26060);
#20834=LINE('',#181305,#26061);
#20835=LINE('',#181312,#26062);
#20836=LINE('',#181315,#26063);
#20837=LINE('',#181318,#26064);
#20838=LINE('',#181324,#26065);
#20839=LINE('',#181327,#26066);
#20840=LINE('',#181333,#26067);
#20841=LINE('',#181340,#26068);
#20842=LINE('',#181343,#26069);
#20843=LINE('',#181346,#26070);
#20844=LINE('',#181364,#26071);
#20845=LINE('',#181371,#26072);
#20846=LINE('',#181374,#26073);
#20847=LINE('',#181377,#26074);
#20848=LINE('',#181383,#26075);
#20849=LINE('',#181386,#26076);
#20850=LINE('',#181392,#26077);
#20851=LINE('',#181399,#26078);
#20852=LINE('',#181402,#26079);
#20853=LINE('',#181405,#26080);
#20854=LINE('',#181423,#26081);
#20855=LINE('',#181430,#26082);
#20856=LINE('',#181433,#26083);
#20857=LINE('',#181436,#26084);
#20858=LINE('',#181442,#26085);
#20859=LINE('',#181445,#26086);
#20860=LINE('',#181451,#26087);
#20861=LINE('',#181458,#26088);
#20862=LINE('',#181461,#26089);
#20863=LINE('',#181464,#26090);
#20864=LINE('',#181482,#26091);
#20865=LINE('',#181489,#26092);
#20866=LINE('',#181492,#26093);
#20867=LINE('',#181495,#26094);
#20868=LINE('',#181501,#26095);
#20869=LINE('',#181504,#26096);
#20870=LINE('',#181510,#26097);
#20871=LINE('',#181517,#26098);
#20872=LINE('',#181520,#26099);
#20873=LINE('',#181523,#26100);
#20874=LINE('',#181541,#26101);
#20875=LINE('',#181548,#26102);
#20876=LINE('',#181551,#26103);
#20877=LINE('',#181554,#26104);
#20878=LINE('',#181560,#26105);
#20879=LINE('',#181563,#26106);
#20880=LINE('',#181569,#26107);
#20881=LINE('',#181576,#26108);
#20882=LINE('',#181579,#26109);
#20883=LINE('',#181582,#26110);
#20884=LINE('',#181600,#26111);
#20885=LINE('',#181607,#26112);
#20886=LINE('',#181610,#26113);
#20887=LINE('',#181613,#26114);
#20888=LINE('',#181619,#26115);
#20889=LINE('',#181622,#26116);
#20890=LINE('',#181628,#26117);
#20891=LINE('',#181635,#26118);
#20892=LINE('',#181638,#26119);
#20893=LINE('',#181641,#26120);
#20894=LINE('',#181659,#26121);
#20895=LINE('',#181666,#26122);
#20896=LINE('',#181669,#26123);
#20897=LINE('',#181672,#26124);
#20898=LINE('',#181678,#26125);
#20899=LINE('',#181681,#26126);
#20900=LINE('',#181687,#26127);
#20901=LINE('',#181694,#26128);
#20902=LINE('',#181697,#26129);
#20903=LINE('',#181700,#26130);
#20904=LINE('',#181718,#26131);
#20905=LINE('',#181725,#26132);
#20906=LINE('',#181728,#26133);
#20907=LINE('',#181731,#26134);
#20908=LINE('',#181737,#26135);
#20909=LINE('',#181740,#26136);
#20910=LINE('',#181746,#26137);
#20911=LINE('',#181753,#26138);
#20912=LINE('',#181756,#26139);
#20913=LINE('',#181759,#26140);
#20914=LINE('',#181777,#26141);
#20915=LINE('',#181784,#26142);
#20916=LINE('',#181787,#26143);
#20917=LINE('',#181790,#26144);
#20918=LINE('',#181796,#26145);
#20919=LINE('',#181799,#26146);
#20920=LINE('',#181805,#26147);
#20921=LINE('',#181812,#26148);
#20922=LINE('',#181815,#26149);
#20923=LINE('',#181818,#26150);
#20924=LINE('',#181836,#26151);
#20925=LINE('',#181843,#26152);
#20926=LINE('',#181846,#26153);
#20927=LINE('',#181849,#26154);
#20928=LINE('',#181855,#26155);
#20929=LINE('',#181858,#26156);
#20930=LINE('',#181864,#26157);
#20931=LINE('',#181871,#26158);
#20932=LINE('',#181874,#26159);
#20933=LINE('',#181877,#26160);
#20934=LINE('',#181895,#26161);
#20935=LINE('',#181902,#26162);
#20936=LINE('',#181905,#26163);
#20937=LINE('',#181908,#26164);
#20938=LINE('',#181914,#26165);
#20939=LINE('',#181917,#26166);
#20940=LINE('',#181923,#26167);
#20941=LINE('',#181930,#26168);
#20942=LINE('',#181933,#26169);
#20943=LINE('',#181936,#26170);
#20944=LINE('',#181955,#26171);
#20945=LINE('',#181962,#26172);
#20946=LINE('',#181965,#26173);
#20947=LINE('',#181968,#26174);
#20948=LINE('',#181974,#26175);
#20949=LINE('',#181977,#26176);
#20950=LINE('',#181983,#26177);
#20951=LINE('',#181990,#26178);
#20952=LINE('',#181993,#26179);
#20953=LINE('',#181996,#26180);
#20954=LINE('',#182014,#26181);
#20955=LINE('',#182018,#26182);
#20956=LINE('',#182025,#26183);
#20957=LINE('',#182027,#26184);
#20958=LINE('',#182029,#26185);
#20959=LINE('',#182033,#26186);
#20960=LINE('',#182035,#26187);
#20961=LINE('',#182039,#26188);
#20962=LINE('',#182043,#26189);
#20963=LINE('',#182044,#26190);
#20964=LINE('',#182050,#26191);
#20965=LINE('',#182052,#26192);
#20966=LINE('',#182054,#26193);
#20967=LINE('',#182058,#26194);
#20968=LINE('',#182060,#26195);
#20969=LINE('',#182064,#26196);
#20970=LINE('',#182068,#26197);
#20971=LINE('',#182069,#26198);
#20972=LINE('',#182489,#26199);
#20973=LINE('',#182493,#26200);
#20974=LINE('',#182500,#26201);
#20975=LINE('',#182502,#26202);
#20976=LINE('',#182504,#26203);
#20977=LINE('',#182508,#26204);
#20978=LINE('',#182510,#26205);
#20979=LINE('',#182514,#26206);
#20980=LINE('',#182518,#26207);
#20981=LINE('',#182519,#26208);
#20982=LINE('',#182525,#26209);
#20983=LINE('',#182527,#26210);
#20984=LINE('',#182529,#26211);
#20985=LINE('',#182533,#26212);
#20986=LINE('',#182535,#26213);
#20987=LINE('',#182539,#26214);
#20988=LINE('',#182543,#26215);
#20989=LINE('',#182544,#26216);
#20990=LINE('',#182548,#26217);
#20991=LINE('',#182552,#26218);
#20992=LINE('',#182559,#26219);
#20993=LINE('',#182561,#26220);
#20994=LINE('',#182563,#26221);
#20995=LINE('',#182567,#26222);
#20996=LINE('',#182569,#26223);
#20997=LINE('',#182573,#26224);
#20998=LINE('',#182577,#26225);
#20999=LINE('',#182578,#26226);
#21000=LINE('',#182584,#26227);
#21001=LINE('',#182586,#26228);
#21002=LINE('',#182588,#26229);
#21003=LINE('',#182592,#26230);
#21004=LINE('',#182594,#26231);
#21005=LINE('',#182598,#26232);
#21006=LINE('',#182602,#26233);
#21007=LINE('',#182603,#26234);
#21008=LINE('',#182607,#26235);
#21009=LINE('',#182611,#26236);
#21010=LINE('',#182618,#26237);
#21011=LINE('',#182620,#26238);
#21012=LINE('',#182622,#26239);
#21013=LINE('',#182626,#26240);
#21014=LINE('',#182628,#26241);
#21015=LINE('',#182632,#26242);
#21016=LINE('',#182636,#26243);
#21017=LINE('',#182637,#26244);
#21018=LINE('',#182643,#26245);
#21019=LINE('',#182645,#26246);
#21020=LINE('',#182647,#26247);
#21021=LINE('',#182651,#26248);
#21022=LINE('',#182653,#26249);
#21023=LINE('',#182657,#26250);
#21024=LINE('',#182661,#26251);
#21025=LINE('',#182662,#26252);
#21026=LINE('',#182666,#26253);
#21027=LINE('',#182670,#26254);
#21028=LINE('',#182677,#26255);
#21029=LINE('',#182679,#26256);
#21030=LINE('',#182681,#26257);
#21031=LINE('',#182685,#26258);
#21032=LINE('',#182687,#26259);
#21033=LINE('',#182691,#26260);
#21034=LINE('',#182695,#26261);
#21035=LINE('',#182696,#26262);
#21036=LINE('',#182702,#26263);
#21037=LINE('',#182704,#26264);
#21038=LINE('',#182706,#26265);
#21039=LINE('',#182710,#26266);
#21040=LINE('',#182712,#26267);
#21041=LINE('',#182716,#26268);
#21042=LINE('',#182720,#26269);
#21043=LINE('',#182721,#26270);
#21044=LINE('',#182725,#26271);
#21045=LINE('',#182729,#26272);
#21046=LINE('',#182736,#26273);
#21047=LINE('',#182738,#26274);
#21048=LINE('',#182740,#26275);
#21049=LINE('',#182744,#26276);
#21050=LINE('',#182746,#26277);
#21051=LINE('',#182750,#26278);
#21052=LINE('',#182754,#26279);
#21053=LINE('',#182755,#26280);
#21054=LINE('',#182761,#26281);
#21055=LINE('',#182763,#26282);
#21056=LINE('',#182765,#26283);
#21057=LINE('',#182769,#26284);
#21058=LINE('',#182771,#26285);
#21059=LINE('',#182775,#26286);
#21060=LINE('',#182779,#26287);
#21061=LINE('',#182780,#26288);
#21062=LINE('',#182784,#26289);
#21063=LINE('',#182788,#26290);
#21064=LINE('',#182795,#26291);
#21065=LINE('',#182797,#26292);
#21066=LINE('',#182799,#26293);
#21067=LINE('',#182803,#26294);
#21068=LINE('',#182805,#26295);
#21069=LINE('',#182809,#26296);
#21070=LINE('',#182813,#26297);
#21071=LINE('',#182814,#26298);
#21072=LINE('',#182820,#26299);
#21073=LINE('',#182822,#26300);
#21074=LINE('',#182824,#26301);
#21075=LINE('',#182828,#26302);
#21076=LINE('',#182830,#26303);
#21077=LINE('',#182834,#26304);
#21078=LINE('',#182838,#26305);
#21079=LINE('',#182839,#26306);
#21080=LINE('',#182843,#26307);
#21081=LINE('',#182847,#26308);
#21082=LINE('',#182854,#26309);
#21083=LINE('',#182856,#26310);
#21084=LINE('',#182858,#26311);
#21085=LINE('',#182862,#26312);
#21086=LINE('',#182864,#26313);
#21087=LINE('',#182868,#26314);
#21088=LINE('',#182872,#26315);
#21089=LINE('',#182873,#26316);
#21090=LINE('',#182879,#26317);
#21091=LINE('',#182881,#26318);
#21092=LINE('',#182883,#26319);
#21093=LINE('',#182887,#26320);
#21094=LINE('',#182889,#26321);
#21095=LINE('',#182893,#26322);
#21096=LINE('',#182897,#26323);
#21097=LINE('',#182898,#26324);
#21098=LINE('',#182902,#26325);
#21099=LINE('',#182906,#26326);
#21100=LINE('',#182913,#26327);
#21101=LINE('',#182915,#26328);
#21102=LINE('',#182917,#26329);
#21103=LINE('',#182921,#26330);
#21104=LINE('',#182923,#26331);
#21105=LINE('',#182927,#26332);
#21106=LINE('',#182931,#26333);
#21107=LINE('',#182932,#26334);
#21108=LINE('',#182938,#26335);
#21109=LINE('',#182940,#26336);
#21110=LINE('',#182942,#26337);
#21111=LINE('',#182946,#26338);
#21112=LINE('',#182948,#26339);
#21113=LINE('',#182952,#26340);
#21114=LINE('',#182956,#26341);
#21115=LINE('',#182957,#26342);
#21116=LINE('',#182961,#26343);
#21117=LINE('',#182965,#26344);
#21118=LINE('',#182972,#26345);
#21119=LINE('',#182974,#26346);
#21120=LINE('',#182976,#26347);
#21121=LINE('',#182980,#26348);
#21122=LINE('',#182982,#26349);
#21123=LINE('',#182986,#26350);
#21124=LINE('',#182990,#26351);
#21125=LINE('',#182991,#26352);
#21126=LINE('',#182997,#26353);
#21127=LINE('',#182999,#26354);
#21128=LINE('',#183001,#26355);
#21129=LINE('',#183005,#26356);
#21130=LINE('',#183007,#26357);
#21131=LINE('',#183011,#26358);
#21132=LINE('',#183015,#26359);
#21133=LINE('',#183016,#26360);
#21134=LINE('',#183020,#26361);
#21135=LINE('',#183024,#26362);
#21136=LINE('',#183031,#26363);
#21137=LINE('',#183033,#26364);
#21138=LINE('',#183035,#26365);
#21139=LINE('',#183039,#26366);
#21140=LINE('',#183041,#26367);
#21141=LINE('',#183045,#26368);
#21142=LINE('',#183049,#26369);
#21143=LINE('',#183050,#26370);
#21144=LINE('',#183056,#26371);
#21145=LINE('',#183058,#26372);
#21146=LINE('',#183060,#26373);
#21147=LINE('',#183064,#26374);
#21148=LINE('',#183066,#26375);
#21149=LINE('',#183070,#26376);
#21150=LINE('',#183074,#26377);
#21151=LINE('',#183075,#26378);
#21152=LINE('',#183079,#26379);
#21153=LINE('',#183083,#26380);
#21154=LINE('',#183090,#26381);
#21155=LINE('',#183092,#26382);
#21156=LINE('',#183094,#26383);
#21157=LINE('',#183098,#26384);
#21158=LINE('',#183100,#26385);
#21159=LINE('',#183104,#26386);
#21160=LINE('',#183108,#26387);
#21161=LINE('',#183109,#26388);
#21162=LINE('',#183115,#26389);
#21163=LINE('',#183117,#26390);
#21164=LINE('',#183119,#26391);
#21165=LINE('',#183123,#26392);
#21166=LINE('',#183125,#26393);
#21167=LINE('',#183129,#26394);
#21168=LINE('',#183133,#26395);
#21169=LINE('',#183134,#26396);
#21170=LINE('',#183138,#26397);
#21171=LINE('',#183142,#26398);
#21172=LINE('',#183149,#26399);
#21173=LINE('',#183151,#26400);
#21174=LINE('',#183153,#26401);
#21175=LINE('',#183157,#26402);
#21176=LINE('',#183159,#26403);
#21177=LINE('',#183163,#26404);
#21178=LINE('',#183167,#26405);
#21179=LINE('',#183168,#26406);
#21180=LINE('',#183174,#26407);
#21181=LINE('',#183176,#26408);
#21182=LINE('',#183178,#26409);
#21183=LINE('',#183182,#26410);
#21184=LINE('',#183184,#26411);
#21185=LINE('',#183188,#26412);
#21186=LINE('',#183192,#26413);
#21187=LINE('',#183193,#26414);
#21188=LINE('',#183197,#26415);
#21189=LINE('',#183201,#26416);
#21190=LINE('',#183208,#26417);
#21191=LINE('',#183210,#26418);
#21192=LINE('',#183212,#26419);
#21193=LINE('',#183216,#26420);
#21194=LINE('',#183218,#26421);
#21195=LINE('',#183222,#26422);
#21196=LINE('',#183226,#26423);
#21197=LINE('',#183227,#26424);
#21198=LINE('',#183233,#26425);
#21199=LINE('',#183235,#26426);
#21200=LINE('',#183237,#26427);
#21201=LINE('',#183241,#26428);
#21202=LINE('',#183243,#26429);
#21203=LINE('',#183247,#26430);
#21204=LINE('',#183251,#26431);
#21205=LINE('',#183252,#26432);
#21206=LINE('',#183256,#26433);
#21207=LINE('',#183260,#26434);
#21208=LINE('',#183267,#26435);
#21209=LINE('',#183269,#26436);
#21210=LINE('',#183271,#26437);
#21211=LINE('',#183275,#26438);
#21212=LINE('',#183277,#26439);
#21213=LINE('',#183281,#26440);
#21214=LINE('',#183285,#26441);
#21215=LINE('',#183286,#26442);
#21216=LINE('',#183292,#26443);
#21217=LINE('',#183294,#26444);
#21218=LINE('',#183296,#26445);
#21219=LINE('',#183300,#26446);
#21220=LINE('',#183302,#26447);
#21221=LINE('',#183306,#26448);
#21222=LINE('',#183310,#26449);
#21223=LINE('',#183311,#26450);
#21224=LINE('',#183315,#26451);
#21225=LINE('',#183319,#26452);
#21226=LINE('',#183326,#26453);
#21227=LINE('',#183328,#26454);
#21228=LINE('',#183330,#26455);
#21229=LINE('',#183334,#26456);
#21230=LINE('',#183336,#26457);
#21231=LINE('',#183340,#26458);
#21232=LINE('',#183344,#26459);
#21233=LINE('',#183345,#26460);
#21234=LINE('',#183351,#26461);
#21235=LINE('',#183353,#26462);
#21236=LINE('',#183355,#26463);
#21237=LINE('',#183359,#26464);
#21238=LINE('',#183361,#26465);
#21239=LINE('',#183365,#26466);
#21240=LINE('',#183369,#26467);
#21241=LINE('',#183370,#26468);
#21242=LINE('',#183374,#26469);
#21243=LINE('',#183378,#26470);
#21244=LINE('',#183385,#26471);
#21245=LINE('',#183387,#26472);
#21246=LINE('',#183389,#26473);
#21247=LINE('',#183393,#26474);
#21248=LINE('',#183395,#26475);
#21249=LINE('',#183399,#26476);
#21250=LINE('',#183403,#26477);
#21251=LINE('',#183404,#26478);
#21252=LINE('',#183410,#26479);
#21253=LINE('',#183412,#26480);
#21254=LINE('',#183414,#26481);
#21255=LINE('',#183418,#26482);
#21256=LINE('',#183420,#26483);
#21257=LINE('',#183424,#26484);
#21258=LINE('',#183428,#26485);
#21259=LINE('',#183429,#26486);
#21260=LINE('',#183433,#26487);
#21261=LINE('',#183437,#26488);
#21262=LINE('',#183444,#26489);
#21263=LINE('',#183446,#26490);
#21264=LINE('',#183448,#26491);
#21265=LINE('',#183452,#26492);
#21266=LINE('',#183454,#26493);
#21267=LINE('',#183458,#26494);
#21268=LINE('',#183462,#26495);
#21269=LINE('',#183463,#26496);
#21270=LINE('',#183469,#26497);
#21271=LINE('',#183471,#26498);
#21272=LINE('',#183473,#26499);
#21273=LINE('',#183477,#26500);
#21274=LINE('',#183479,#26501);
#21275=LINE('',#183483,#26502);
#21276=LINE('',#183487,#26503);
#21277=LINE('',#183488,#26504);
#21278=LINE('',#183492,#26505);
#21279=LINE('',#183496,#26506);
#21280=LINE('',#183503,#26507);
#21281=LINE('',#183505,#26508);
#21282=LINE('',#183507,#26509);
#21283=LINE('',#183511,#26510);
#21284=LINE('',#183513,#26511);
#21285=LINE('',#183517,#26512);
#21286=LINE('',#183521,#26513);
#21287=LINE('',#183522,#26514);
#21288=LINE('',#183528,#26515);
#21289=LINE('',#183530,#26516);
#21290=LINE('',#183532,#26517);
#21291=LINE('',#183536,#26518);
#21292=LINE('',#183538,#26519);
#21293=LINE('',#183542,#26520);
#21294=LINE('',#183546,#26521);
#21295=LINE('',#183547,#26522);
#21296=LINE('',#183551,#26523);
#21297=LINE('',#183555,#26524);
#21298=LINE('',#183562,#26525);
#21299=LINE('',#183564,#26526);
#21300=LINE('',#183566,#26527);
#21301=LINE('',#183570,#26528);
#21302=LINE('',#183572,#26529);
#21303=LINE('',#183576,#26530);
#21304=LINE('',#183580,#26531);
#21305=LINE('',#183581,#26532);
#21306=LINE('',#183587,#26533);
#21307=LINE('',#183589,#26534);
#21308=LINE('',#183591,#26535);
#21309=LINE('',#183595,#26536);
#21310=LINE('',#183597,#26537);
#21311=LINE('',#183601,#26538);
#21312=LINE('',#183605,#26539);
#21313=LINE('',#183606,#26540);
#21314=LINE('',#183610,#26541);
#21315=LINE('',#183614,#26542);
#21316=LINE('',#183621,#26543);
#21317=LINE('',#183623,#26544);
#21318=LINE('',#183625,#26545);
#21319=LINE('',#183629,#26546);
#21320=LINE('',#183631,#26547);
#21321=LINE('',#183635,#26548);
#21322=LINE('',#183639,#26549);
#21323=LINE('',#183640,#26550);
#21324=LINE('',#183646,#26551);
#21325=LINE('',#183648,#26552);
#21326=LINE('',#183650,#26553);
#21327=LINE('',#183654,#26554);
#21328=LINE('',#183656,#26555);
#21329=LINE('',#183660,#26556);
#21330=LINE('',#183664,#26557);
#21331=LINE('',#183665,#26558);
#21332=LINE('',#183669,#26559);
#21333=LINE('',#183673,#26560);
#21334=LINE('',#183680,#26561);
#21335=LINE('',#183682,#26562);
#21336=LINE('',#183684,#26563);
#21337=LINE('',#183688,#26564);
#21338=LINE('',#183690,#26565);
#21339=LINE('',#183694,#26566);
#21340=LINE('',#183698,#26567);
#21341=LINE('',#183699,#26568);
#21342=LINE('',#183705,#26569);
#21343=LINE('',#183707,#26570);
#21344=LINE('',#183709,#26571);
#21345=LINE('',#183713,#26572);
#21346=LINE('',#183715,#26573);
#21347=LINE('',#183719,#26574);
#21348=LINE('',#183723,#26575);
#21349=LINE('',#183724,#26576);
#21350=LINE('',#183728,#26577);
#21351=LINE('',#183732,#26578);
#21352=LINE('',#183739,#26579);
#21353=LINE('',#183741,#26580);
#21354=LINE('',#183743,#26581);
#21355=LINE('',#183747,#26582);
#21356=LINE('',#183749,#26583);
#21357=LINE('',#183753,#26584);
#21358=LINE('',#183757,#26585);
#21359=LINE('',#183758,#26586);
#21360=LINE('',#183764,#26587);
#21361=LINE('',#183766,#26588);
#21362=LINE('',#183768,#26589);
#21363=LINE('',#183772,#26590);
#21364=LINE('',#183774,#26591);
#21365=LINE('',#183778,#26592);
#21366=LINE('',#183782,#26593);
#21367=LINE('',#183783,#26594);
#21368=LINE('',#183787,#26595);
#21369=LINE('',#183791,#26596);
#21370=LINE('',#183798,#26597);
#21371=LINE('',#183800,#26598);
#21372=LINE('',#183802,#26599);
#21373=LINE('',#183806,#26600);
#21374=LINE('',#183808,#26601);
#21375=LINE('',#183812,#26602);
#21376=LINE('',#183816,#26603);
#21377=LINE('',#183817,#26604);
#21378=LINE('',#183823,#26605);
#21379=LINE('',#183825,#26606);
#21380=LINE('',#183827,#26607);
#21381=LINE('',#183831,#26608);
#21382=LINE('',#183833,#26609);
#21383=LINE('',#183837,#26610);
#21384=LINE('',#183841,#26611);
#21385=LINE('',#183842,#26612);
#21386=LINE('',#183846,#26613);
#21387=LINE('',#183850,#26614);
#21388=LINE('',#183857,#26615);
#21389=LINE('',#183859,#26616);
#21390=LINE('',#183861,#26617);
#21391=LINE('',#183865,#26618);
#21392=LINE('',#183867,#26619);
#21393=LINE('',#183871,#26620);
#21394=LINE('',#183875,#26621);
#21395=LINE('',#183876,#26622);
#21396=LINE('',#183882,#26623);
#21397=LINE('',#183884,#26624);
#21398=LINE('',#183886,#26625);
#21399=LINE('',#183890,#26626);
#21400=LINE('',#183892,#26627);
#21401=LINE('',#183896,#26628);
#21402=LINE('',#183900,#26629);
#21403=LINE('',#183901,#26630);
#21404=LINE('',#183905,#26631);
#21405=LINE('',#183909,#26632);
#21406=LINE('',#183916,#26633);
#21407=LINE('',#183918,#26634);
#21408=LINE('',#183920,#26635);
#21409=LINE('',#183924,#26636);
#21410=LINE('',#183926,#26637);
#21411=LINE('',#183930,#26638);
#21412=LINE('',#183934,#26639);
#21413=LINE('',#183935,#26640);
#21414=LINE('',#183941,#26641);
#21415=LINE('',#183943,#26642);
#21416=LINE('',#183945,#26643);
#21417=LINE('',#183949,#26644);
#21418=LINE('',#183951,#26645);
#21419=LINE('',#183955,#26646);
#21420=LINE('',#183959,#26647);
#21421=LINE('',#183960,#26648);
#21422=LINE('',#183964,#26649);
#21423=LINE('',#183968,#26650);
#21424=LINE('',#183975,#26651);
#21425=LINE('',#183977,#26652);
#21426=LINE('',#183979,#26653);
#21427=LINE('',#183983,#26654);
#21428=LINE('',#183985,#26655);
#21429=LINE('',#183989,#26656);
#21430=LINE('',#183993,#26657);
#21431=LINE('',#183994,#26658);
#21432=LINE('',#184000,#26659);
#21433=LINE('',#184002,#26660);
#21434=LINE('',#184004,#26661);
#21435=LINE('',#184008,#26662);
#21436=LINE('',#184010,#26663);
#21437=LINE('',#184014,#26664);
#21438=LINE('',#184018,#26665);
#21439=LINE('',#184019,#26666);
#21440=LINE('',#184023,#26667);
#21441=LINE('',#184027,#26668);
#21442=LINE('',#184034,#26669);
#21443=LINE('',#184036,#26670);
#21444=LINE('',#184038,#26671);
#21445=LINE('',#184042,#26672);
#21446=LINE('',#184044,#26673);
#21447=LINE('',#184048,#26674);
#21448=LINE('',#184052,#26675);
#21449=LINE('',#184053,#26676);
#21450=LINE('',#184059,#26677);
#21451=LINE('',#184061,#26678);
#21452=LINE('',#184063,#26679);
#21453=LINE('',#184067,#26680);
#21454=LINE('',#184069,#26681);
#21455=LINE('',#184073,#26682);
#21456=LINE('',#184077,#26683);
#21457=LINE('',#184078,#26684);
#21458=LINE('',#184082,#26685);
#21459=LINE('',#184086,#26686);
#21460=LINE('',#184093,#26687);
#21461=LINE('',#184095,#26688);
#21462=LINE('',#184097,#26689);
#21463=LINE('',#184101,#26690);
#21464=LINE('',#184103,#26691);
#21465=LINE('',#184107,#26692);
#21466=LINE('',#184111,#26693);
#21467=LINE('',#184112,#26694);
#21468=LINE('',#184118,#26695);
#21469=LINE('',#184120,#26696);
#21470=LINE('',#184122,#26697);
#21471=LINE('',#184126,#26698);
#21472=LINE('',#184128,#26699);
#21473=LINE('',#184132,#26700);
#21474=LINE('',#184136,#26701);
#21475=LINE('',#184137,#26702);
#21476=LINE('',#184141,#26703);
#21477=LINE('',#184145,#26704);
#21478=LINE('',#184152,#26705);
#21479=LINE('',#184154,#26706);
#21480=LINE('',#184156,#26707);
#21481=LINE('',#184160,#26708);
#21482=LINE('',#184162,#26709);
#21483=LINE('',#184166,#26710);
#21484=LINE('',#184170,#26711);
#21485=LINE('',#184171,#26712);
#21486=LINE('',#184177,#26713);
#21487=LINE('',#184179,#26714);
#21488=LINE('',#184181,#26715);
#21489=LINE('',#184185,#26716);
#21490=LINE('',#184187,#26717);
#21491=LINE('',#184191,#26718);
#21492=LINE('',#184195,#26719);
#21493=LINE('',#184196,#26720);
#21494=LINE('',#184198,#26721);
#21495=LINE('',#184199,#26722);
#21496=LINE('',#184205,#26723);
#21497=LINE('',#184207,#26724);
#21498=LINE('',#184209,#26725);
#21499=LINE('',#184213,#26726);
#21500=LINE('',#184215,#26727);
#21501=LINE('',#184219,#26728);
#21502=LINE('',#184223,#26729);
#21503=LINE('',#184224,#26730);
#21504=LINE('',#184230,#26731);
#21505=LINE('',#184232,#26732);
#21506=LINE('',#184234,#26733);
#21507=LINE('',#184238,#26734);
#21508=LINE('',#184240,#26735);
#21509=LINE('',#184244,#26736);
#21510=LINE('',#184248,#26737);
#21511=LINE('',#184249,#26738);
#21512=LINE('',#184253,#26739);
#21513=LINE('',#184257,#26740);
#21514=LINE('',#184264,#26741);
#21515=LINE('',#184266,#26742);
#21516=LINE('',#184268,#26743);
#21517=LINE('',#184272,#26744);
#21518=LINE('',#184274,#26745);
#21519=LINE('',#184278,#26746);
#21520=LINE('',#184282,#26747);
#21521=LINE('',#184283,#26748);
#21522=LINE('',#184289,#26749);
#21523=LINE('',#184291,#26750);
#21524=LINE('',#184293,#26751);
#21525=LINE('',#184297,#26752);
#21526=LINE('',#184299,#26753);
#21527=LINE('',#184303,#26754);
#21528=LINE('',#184307,#26755);
#21529=LINE('',#184308,#26756);
#21530=LINE('',#184312,#26757);
#21531=LINE('',#184316,#26758);
#21532=LINE('',#184323,#26759);
#21533=LINE('',#184325,#26760);
#21534=LINE('',#184327,#26761);
#21535=LINE('',#184331,#26762);
#21536=LINE('',#184333,#26763);
#21537=LINE('',#184337,#26764);
#21538=LINE('',#184341,#26765);
#21539=LINE('',#184342,#26766);
#21540=LINE('',#184348,#26767);
#21541=LINE('',#184350,#26768);
#21542=LINE('',#184352,#26769);
#21543=LINE('',#184356,#26770);
#21544=LINE('',#184358,#26771);
#21545=LINE('',#184362,#26772);
#21546=LINE('',#184366,#26773);
#21547=LINE('',#184367,#26774);
#21548=LINE('',#184371,#26775);
#21549=LINE('',#184375,#26776);
#21550=LINE('',#184382,#26777);
#21551=LINE('',#184384,#26778);
#21552=LINE('',#184386,#26779);
#21553=LINE('',#184390,#26780);
#21554=LINE('',#184392,#26781);
#21555=LINE('',#184396,#26782);
#21556=LINE('',#184400,#26783);
#21557=LINE('',#184401,#26784);
#21558=LINE('',#184407,#26785);
#21559=LINE('',#184409,#26786);
#21560=LINE('',#184411,#26787);
#21561=LINE('',#184415,#26788);
#21562=LINE('',#184417,#26789);
#21563=LINE('',#184421,#26790);
#21564=LINE('',#184425,#26791);
#21565=LINE('',#184426,#26792);
#21566=LINE('',#184430,#26793);
#21567=LINE('',#184434,#26794);
#21568=LINE('',#184441,#26795);
#21569=LINE('',#184443,#26796);
#21570=LINE('',#184445,#26797);
#21571=LINE('',#184449,#26798);
#21572=LINE('',#184451,#26799);
#21573=LINE('',#184455,#26800);
#21574=LINE('',#184459,#26801);
#21575=LINE('',#184460,#26802);
#21576=LINE('',#184466,#26803);
#21577=LINE('',#184468,#26804);
#21578=LINE('',#184470,#26805);
#21579=LINE('',#184474,#26806);
#21580=LINE('',#184476,#26807);
#21581=LINE('',#184480,#26808);
#21582=LINE('',#184484,#26809);
#21583=LINE('',#184485,#26810);
#21584=LINE('',#184489,#26811);
#21585=LINE('',#184493,#26812);
#21586=LINE('',#184500,#26813);
#21587=LINE('',#184502,#26814);
#21588=LINE('',#184504,#26815);
#21589=LINE('',#184508,#26816);
#21590=LINE('',#184510,#26817);
#21591=LINE('',#184514,#26818);
#21592=LINE('',#184518,#26819);
#21593=LINE('',#184519,#26820);
#21594=LINE('',#184525,#26821);
#21595=LINE('',#184527,#26822);
#21596=LINE('',#184529,#26823);
#21597=LINE('',#184533,#26824);
#21598=LINE('',#184535,#26825);
#21599=LINE('',#184539,#26826);
#21600=LINE('',#184543,#26827);
#21601=LINE('',#184544,#26828);
#21602=LINE('',#184548,#26829);
#21603=LINE('',#184552,#26830);
#21604=LINE('',#184559,#26831);
#21605=LINE('',#184561,#26832);
#21606=LINE('',#184563,#26833);
#21607=LINE('',#184567,#26834);
#21608=LINE('',#184569,#26835);
#21609=LINE('',#184573,#26836);
#21610=LINE('',#184577,#26837);
#21611=LINE('',#184578,#26838);
#21612=LINE('',#184584,#26839);
#21613=LINE('',#184586,#26840);
#21614=LINE('',#184588,#26841);
#21615=LINE('',#184592,#26842);
#21616=LINE('',#184594,#26843);
#21617=LINE('',#184598,#26844);
#21618=LINE('',#184602,#26845);
#21619=LINE('',#184603,#26846);
#21620=LINE('',#184607,#26847);
#21621=LINE('',#184611,#26848);
#21622=LINE('',#184618,#26849);
#21623=LINE('',#184620,#26850);
#21624=LINE('',#184622,#26851);
#21625=LINE('',#184626,#26852);
#21626=LINE('',#184628,#26853);
#21627=LINE('',#184632,#26854);
#21628=LINE('',#184636,#26855);
#21629=LINE('',#184637,#26856);
#21630=LINE('',#184643,#26857);
#21631=LINE('',#184645,#26858);
#21632=LINE('',#184647,#26859);
#21633=LINE('',#184651,#26860);
#21634=LINE('',#184653,#26861);
#21635=LINE('',#184657,#26862);
#21636=LINE('',#184661,#26863);
#21637=LINE('',#184662,#26864);
#21638=LINE('',#184666,#26865);
#21639=LINE('',#184670,#26866);
#21640=LINE('',#184677,#26867);
#21641=LINE('',#184679,#26868);
#21642=LINE('',#184681,#26869);
#21643=LINE('',#184685,#26870);
#21644=LINE('',#184687,#26871);
#21645=LINE('',#184691,#26872);
#21646=LINE('',#184695,#26873);
#21647=LINE('',#184696,#26874);
#21648=LINE('',#184702,#26875);
#21649=LINE('',#184704,#26876);
#21650=LINE('',#184706,#26877);
#21651=LINE('',#184710,#26878);
#21652=LINE('',#184712,#26879);
#21653=LINE('',#184716,#26880);
#21654=LINE('',#184720,#26881);
#21655=LINE('',#184721,#26882);
#21656=LINE('',#184725,#26883);
#21657=LINE('',#184729,#26884);
#21658=LINE('',#184736,#26885);
#21659=LINE('',#184738,#26886);
#21660=LINE('',#184740,#26887);
#21661=LINE('',#184744,#26888);
#21662=LINE('',#184746,#26889);
#21663=LINE('',#184750,#26890);
#21664=LINE('',#184754,#26891);
#21665=LINE('',#184755,#26892);
#21666=LINE('',#184761,#26893);
#21667=LINE('',#184763,#26894);
#21668=LINE('',#184765,#26895);
#21669=LINE('',#184769,#26896);
#21670=LINE('',#184771,#26897);
#21671=LINE('',#184775,#26898);
#21672=LINE('',#184779,#26899);
#21673=LINE('',#184780,#26900);
#21674=LINE('',#184784,#26901);
#21675=LINE('',#184788,#26902);
#21676=LINE('',#184795,#26903);
#21677=LINE('',#184797,#26904);
#21678=LINE('',#184799,#26905);
#21679=LINE('',#184803,#26906);
#21680=LINE('',#184805,#26907);
#21681=LINE('',#184809,#26908);
#21682=LINE('',#184813,#26909);
#21683=LINE('',#184814,#26910);
#21684=LINE('',#184820,#26911);
#21685=LINE('',#184822,#26912);
#21686=LINE('',#184824,#26913);
#21687=LINE('',#184828,#26914);
#21688=LINE('',#184830,#26915);
#21689=LINE('',#184834,#26916);
#21690=LINE('',#184838,#26917);
#21691=LINE('',#184839,#26918);
#21692=LINE('',#184843,#26919);
#21693=LINE('',#184847,#26920);
#21694=LINE('',#184854,#26921);
#21695=LINE('',#184856,#26922);
#21696=LINE('',#184858,#26923);
#21697=LINE('',#184862,#26924);
#21698=LINE('',#184864,#26925);
#21699=LINE('',#184868,#26926);
#21700=LINE('',#184872,#26927);
#21701=LINE('',#184873,#26928);
#21702=LINE('',#184879,#26929);
#21703=LINE('',#184881,#26930);
#21704=LINE('',#184883,#26931);
#21705=LINE('',#184887,#26932);
#21706=LINE('',#184889,#26933);
#21707=LINE('',#184893,#26934);
#21708=LINE('',#184897,#26935);
#21709=LINE('',#184898,#26936);
#21710=LINE('',#184902,#26937);
#21711=LINE('',#184906,#26938);
#21712=LINE('',#184913,#26939);
#21713=LINE('',#184915,#26940);
#21714=LINE('',#184917,#26941);
#21715=LINE('',#184921,#26942);
#21716=LINE('',#184923,#26943);
#21717=LINE('',#184927,#26944);
#21718=LINE('',#184931,#26945);
#21719=LINE('',#184932,#26946);
#21720=LINE('',#184938,#26947);
#21721=LINE('',#184940,#26948);
#21722=LINE('',#184942,#26949);
#21723=LINE('',#184946,#26950);
#21724=LINE('',#184948,#26951);
#21725=LINE('',#184952,#26952);
#21726=LINE('',#184956,#26953);
#21727=LINE('',#184957,#26954);
#21728=LINE('',#184961,#26955);
#21729=LINE('',#184965,#26956);
#21730=LINE('',#184972,#26957);
#21731=LINE('',#184974,#26958);
#21732=LINE('',#184976,#26959);
#21733=LINE('',#184980,#26960);
#21734=LINE('',#184982,#26961);
#21735=LINE('',#184986,#26962);
#21736=LINE('',#184990,#26963);
#21737=LINE('',#184991,#26964);
#21738=LINE('',#184997,#26965);
#21739=LINE('',#184999,#26966);
#21740=LINE('',#185001,#26967);
#21741=LINE('',#185005,#26968);
#21742=LINE('',#185007,#26969);
#21743=LINE('',#185011,#26970);
#21744=LINE('',#185015,#26971);
#21745=LINE('',#185016,#26972);
#21746=LINE('',#185020,#26973);
#21747=LINE('',#185024,#26974);
#21748=LINE('',#185031,#26975);
#21749=LINE('',#185033,#26976);
#21750=LINE('',#185035,#26977);
#21751=LINE('',#185039,#26978);
#21752=LINE('',#185041,#26979);
#21753=LINE('',#185045,#26980);
#21754=LINE('',#185049,#26981);
#21755=LINE('',#185050,#26982);
#21756=LINE('',#185056,#26983);
#21757=LINE('',#185058,#26984);
#21758=LINE('',#185060,#26985);
#21759=LINE('',#185064,#26986);
#21760=LINE('',#185066,#26987);
#21761=LINE('',#185070,#26988);
#21762=LINE('',#185074,#26989);
#21763=LINE('',#185075,#26990);
#21764=LINE('',#185077,#26991);
#21765=LINE('',#185078,#26992);
#21766=LINE('',#185084,#26993);
#21767=LINE('',#185086,#26994);
#21768=LINE('',#185088,#26995);
#21769=LINE('',#185092,#26996);
#21770=LINE('',#185094,#26997);
#21771=LINE('',#185098,#26998);
#21772=LINE('',#185102,#26999);
#21773=LINE('',#185103,#27000);
#21774=LINE('',#185109,#27001);
#21775=LINE('',#185111,#27002);
#21776=LINE('',#185113,#27003);
#21777=LINE('',#185117,#27004);
#21778=LINE('',#185119,#27005);
#21779=LINE('',#185123,#27006);
#21780=LINE('',#185127,#27007);
#21781=LINE('',#185128,#27008);
#21782=LINE('',#185132,#27009);
#21783=LINE('',#185136,#27010);
#21784=LINE('',#185143,#27011);
#21785=LINE('',#185145,#27012);
#21786=LINE('',#185147,#27013);
#21787=LINE('',#185151,#27014);
#21788=LINE('',#185153,#27015);
#21789=LINE('',#185157,#27016);
#21790=LINE('',#185161,#27017);
#21791=LINE('',#185162,#27018);
#21792=LINE('',#185168,#27019);
#21793=LINE('',#185170,#27020);
#21794=LINE('',#185172,#27021);
#21795=LINE('',#185176,#27022);
#21796=LINE('',#185178,#27023);
#21797=LINE('',#185182,#27024);
#21798=LINE('',#185186,#27025);
#21799=LINE('',#185187,#27026);
#21800=LINE('',#185191,#27027);
#21801=LINE('',#185195,#27028);
#21802=LINE('',#185202,#27029);
#21803=LINE('',#185204,#27030);
#21804=LINE('',#185206,#27031);
#21805=LINE('',#185210,#27032);
#21806=LINE('',#185212,#27033);
#21807=LINE('',#185216,#27034);
#21808=LINE('',#185220,#27035);
#21809=LINE('',#185221,#27036);
#21810=LINE('',#185227,#27037);
#21811=LINE('',#185229,#27038);
#21812=LINE('',#185231,#27039);
#21813=LINE('',#185235,#27040);
#21814=LINE('',#185237,#27041);
#21815=LINE('',#185241,#27042);
#21816=LINE('',#185245,#27043);
#21817=LINE('',#185246,#27044);
#21818=LINE('',#185250,#27045);
#21819=LINE('',#185254,#27046);
#21820=LINE('',#185261,#27047);
#21821=LINE('',#185263,#27048);
#21822=LINE('',#185265,#27049);
#21823=LINE('',#185269,#27050);
#21824=LINE('',#185271,#27051);
#21825=LINE('',#185275,#27052);
#21826=LINE('',#185279,#27053);
#21827=LINE('',#185280,#27054);
#21828=LINE('',#185286,#27055);
#21829=LINE('',#185288,#27056);
#21830=LINE('',#185290,#27057);
#21831=LINE('',#185294,#27058);
#21832=LINE('',#185296,#27059);
#21833=LINE('',#185300,#27060);
#21834=LINE('',#185304,#27061);
#21835=LINE('',#185305,#27062);
#21836=LINE('',#185309,#27063);
#21837=LINE('',#185313,#27064);
#21838=LINE('',#185320,#27065);
#21839=LINE('',#185322,#27066);
#21840=LINE('',#185324,#27067);
#21841=LINE('',#185328,#27068);
#21842=LINE('',#185330,#27069);
#21843=LINE('',#185334,#27070);
#21844=LINE('',#185338,#27071);
#21845=LINE('',#185339,#27072);
#21846=LINE('',#185345,#27073);
#21847=LINE('',#185347,#27074);
#21848=LINE('',#185349,#27075);
#21849=LINE('',#185353,#27076);
#21850=LINE('',#185355,#27077);
#21851=LINE('',#185359,#27078);
#21852=LINE('',#185363,#27079);
#21853=LINE('',#185364,#27080);
#21854=LINE('',#185368,#27081);
#21855=LINE('',#185372,#27082);
#21856=LINE('',#185379,#27083);
#21857=LINE('',#185381,#27084);
#21858=LINE('',#185383,#27085);
#21859=LINE('',#185387,#27086);
#21860=LINE('',#185389,#27087);
#21861=LINE('',#185393,#27088);
#21862=LINE('',#185397,#27089);
#21863=LINE('',#185398,#27090);
#21864=LINE('',#185404,#27091);
#21865=LINE('',#185406,#27092);
#21866=LINE('',#185408,#27093);
#21867=LINE('',#185412,#27094);
#21868=LINE('',#185414,#27095);
#21869=LINE('',#185418,#27096);
#21870=LINE('',#185422,#27097);
#21871=LINE('',#185423,#27098);
#21872=LINE('',#185427,#27099);
#21873=LINE('',#185431,#27100);
#21874=LINE('',#185438,#27101);
#21875=LINE('',#185440,#27102);
#21876=LINE('',#185442,#27103);
#21877=LINE('',#185446,#27104);
#21878=LINE('',#185448,#27105);
#21879=LINE('',#185452,#27106);
#21880=LINE('',#185456,#27107);
#21881=LINE('',#185457,#27108);
#21882=LINE('',#185463,#27109);
#21883=LINE('',#185465,#27110);
#21884=LINE('',#185467,#27111);
#21885=LINE('',#185471,#27112);
#21886=LINE('',#185473,#27113);
#21887=LINE('',#185477,#27114);
#21888=LINE('',#185481,#27115);
#21889=LINE('',#185482,#27116);
#21890=LINE('',#185486,#27117);
#21891=LINE('',#185490,#27118);
#21892=LINE('',#185497,#27119);
#21893=LINE('',#185499,#27120);
#21894=LINE('',#185501,#27121);
#21895=LINE('',#185505,#27122);
#21896=LINE('',#185507,#27123);
#21897=LINE('',#185511,#27124);
#21898=LINE('',#185515,#27125);
#21899=LINE('',#185516,#27126);
#21900=LINE('',#185522,#27127);
#21901=LINE('',#185524,#27128);
#21902=LINE('',#185526,#27129);
#21903=LINE('',#185530,#27130);
#21904=LINE('',#185532,#27131);
#21905=LINE('',#185536,#27132);
#21906=LINE('',#185540,#27133);
#21907=LINE('',#185541,#27134);
#21908=LINE('',#185545,#27135);
#21909=LINE('',#185549,#27136);
#21910=LINE('',#185556,#27137);
#21911=LINE('',#185558,#27138);
#21912=LINE('',#185560,#27139);
#21913=LINE('',#185564,#27140);
#21914=LINE('',#185566,#27141);
#21915=LINE('',#185570,#27142);
#21916=LINE('',#185574,#27143);
#21917=LINE('',#185575,#27144);
#21918=LINE('',#185581,#27145);
#21919=LINE('',#185583,#27146);
#21920=LINE('',#185585,#27147);
#21921=LINE('',#185589,#27148);
#21922=LINE('',#185591,#27149);
#21923=LINE('',#185595,#27150);
#21924=LINE('',#185599,#27151);
#21925=LINE('',#185600,#27152);
#21926=LINE('',#185604,#27153);
#21927=LINE('',#185608,#27154);
#21928=LINE('',#185615,#27155);
#21929=LINE('',#185617,#27156);
#21930=LINE('',#185619,#27157);
#21931=LINE('',#185623,#27158);
#21932=LINE('',#185625,#27159);
#21933=LINE('',#185629,#27160);
#21934=LINE('',#185633,#27161);
#21935=LINE('',#185634,#27162);
#21936=LINE('',#185640,#27163);
#21937=LINE('',#185642,#27164);
#21938=LINE('',#185644,#27165);
#21939=LINE('',#185648,#27166);
#21940=LINE('',#185650,#27167);
#21941=LINE('',#185654,#27168);
#21942=LINE('',#185658,#27169);
#21943=LINE('',#185659,#27170);
#21944=LINE('',#185663,#27171);
#21945=LINE('',#185667,#27172);
#21946=LINE('',#185674,#27173);
#21947=LINE('',#185676,#27174);
#21948=LINE('',#185678,#27175);
#21949=LINE('',#185682,#27176);
#21950=LINE('',#185684,#27177);
#21951=LINE('',#185688,#27178);
#21952=LINE('',#185692,#27179);
#21953=LINE('',#185693,#27180);
#21954=LINE('',#185699,#27181);
#21955=LINE('',#185701,#27182);
#21956=LINE('',#185703,#27183);
#21957=LINE('',#185707,#27184);
#21958=LINE('',#185709,#27185);
#21959=LINE('',#185713,#27186);
#21960=LINE('',#185717,#27187);
#21961=LINE('',#185718,#27188);
#21962=LINE('',#185722,#27189);
#21963=LINE('',#185726,#27190);
#21964=LINE('',#185733,#27191);
#21965=LINE('',#185735,#27192);
#21966=LINE('',#185737,#27193);
#21967=LINE('',#185741,#27194);
#21968=LINE('',#185743,#27195);
#21969=LINE('',#185747,#27196);
#21970=LINE('',#185751,#27197);
#21971=LINE('',#185752,#27198);
#21972=LINE('',#185758,#27199);
#21973=LINE('',#185760,#27200);
#21974=LINE('',#185762,#27201);
#21975=LINE('',#185766,#27202);
#21976=LINE('',#185768,#27203);
#21977=LINE('',#185772,#27204);
#21978=LINE('',#185776,#27205);
#21979=LINE('',#185777,#27206);
#21980=LINE('',#185781,#27207);
#21981=LINE('',#185785,#27208);
#21982=LINE('',#185792,#27209);
#21983=LINE('',#185794,#27210);
#21984=LINE('',#185796,#27211);
#21985=LINE('',#185800,#27212);
#21986=LINE('',#185802,#27213);
#21987=LINE('',#185806,#27214);
#21988=LINE('',#185810,#27215);
#21989=LINE('',#185811,#27216);
#21990=LINE('',#185817,#27217);
#21991=LINE('',#185819,#27218);
#21992=LINE('',#185821,#27219);
#21993=LINE('',#185825,#27220);
#21994=LINE('',#185827,#27221);
#21995=LINE('',#185831,#27222);
#21996=LINE('',#185835,#27223);
#21997=LINE('',#185836,#27224);
#21998=LINE('',#185840,#27225);
#21999=LINE('',#185844,#27226);
#22000=LINE('',#185851,#27227);
#22001=LINE('',#185853,#27228);
#22002=LINE('',#185855,#27229);
#22003=LINE('',#185859,#27230);
#22004=LINE('',#185861,#27231);
#22005=LINE('',#185865,#27232);
#22006=LINE('',#185869,#27233);
#22007=LINE('',#185870,#27234);
#22008=LINE('',#185876,#27235);
#22009=LINE('',#185878,#27236);
#22010=LINE('',#185880,#27237);
#22011=LINE('',#185884,#27238);
#22012=LINE('',#185886,#27239);
#22013=LINE('',#185890,#27240);
#22014=LINE('',#185894,#27241);
#22015=LINE('',#185895,#27242);
#22016=LINE('',#185899,#27243);
#22017=LINE('',#185903,#27244);
#22018=LINE('',#185910,#27245);
#22019=LINE('',#185912,#27246);
#22020=LINE('',#185914,#27247);
#22021=LINE('',#185918,#27248);
#22022=LINE('',#185920,#27249);
#22023=LINE('',#185924,#27250);
#22024=LINE('',#185928,#27251);
#22025=LINE('',#185929,#27252);
#22026=LINE('',#185935,#27253);
#22027=LINE('',#185937,#27254);
#22028=LINE('',#185939,#27255);
#22029=LINE('',#185943,#27256);
#22030=LINE('',#185945,#27257);
#22031=LINE('',#185949,#27258);
#22032=LINE('',#185953,#27259);
#22033=LINE('',#185954,#27260);
#22034=LINE('',#210557,#27261);
#22035=LINE('',#210560,#27262);
#22036=LINE('',#210610,#27263);
#22037=LINE('',#210614,#27264);
#22038=LINE('',#210703,#27265);
#22039=LINE('',#210707,#27266);
#22040=LINE('',#210796,#27267);
#22041=LINE('',#210800,#27268);
#22042=LINE('',#210889,#27269);
#22043=LINE('',#210893,#27270);
#22044=LINE('',#210982,#27271);
#22045=LINE('',#210986,#27272);
#22046=LINE('',#211075,#27273);
#22047=LINE('',#211079,#27274);
#22048=LINE('',#211168,#27275);
#22049=LINE('',#211172,#27276);
#22050=LINE('',#211261,#27277);
#22051=LINE('',#211265,#27278);
#22052=LINE('',#211354,#27279);
#22053=LINE('',#211358,#27280);
#22054=LINE('',#211447,#27281);
#22055=LINE('',#211451,#27282);
#22056=LINE('',#211540,#27283);
#22057=LINE('',#211544,#27284);
#22058=LINE('',#211633,#27285);
#22059=LINE('',#211637,#27286);
#22060=LINE('',#211726,#27287);
#22061=LINE('',#211730,#27288);
#22062=LINE('',#211819,#27289);
#22063=LINE('',#211823,#27290);
#22064=LINE('',#211912,#27291);
#22065=LINE('',#211916,#27292);
#22066=LINE('',#212005,#27293);
#22067=LINE('',#212009,#27294);
#22068=LINE('',#212098,#27295);
#22069=LINE('',#212102,#27296);
#22070=LINE('',#212191,#27297);
#22071=LINE('',#212195,#27298);
#22072=LINE('',#212284,#27299);
#22073=LINE('',#212288,#27300);
#22074=LINE('',#212377,#27301);
#22075=LINE('',#212381,#27302);
#22076=LINE('',#212470,#27303);
#22077=LINE('',#212474,#27304);
#22078=LINE('',#212563,#27305);
#22079=LINE('',#212567,#27306);
#22080=LINE('',#212656,#27307);
#22081=LINE('',#212660,#27308);
#22082=LINE('',#212749,#27309);
#22083=LINE('',#212753,#27310);
#22084=LINE('',#212842,#27311);
#22085=LINE('',#212846,#27312);
#22086=LINE('',#212935,#27313);
#22087=LINE('',#212939,#27314);
#22088=LINE('',#213028,#27315);
#22089=LINE('',#213032,#27316);
#22090=LINE('',#213121,#27317);
#22091=LINE('',#213125,#27318);
#22092=LINE('',#213214,#27319);
#22093=LINE('',#213218,#27320);
#22094=LINE('',#213307,#27321);
#22095=LINE('',#213311,#27322);
#22096=LINE('',#213352,#27323);
#22097=LINE('',#213398,#27324);
#22098=LINE('',#213402,#27325);
#22099=LINE('',#213491,#27326);
#22100=LINE('',#213495,#27327);
#22101=LINE('',#213584,#27328);
#22102=LINE('',#213588,#27329);
#22103=LINE('',#213677,#27330);
#22104=LINE('',#213681,#27331);
#22105=LINE('',#213770,#27332);
#22106=LINE('',#213774,#27333);
#22107=LINE('',#213863,#27334);
#22108=LINE('',#213867,#27335);
#22109=LINE('',#213956,#27336);
#22110=LINE('',#213960,#27337);
#22111=LINE('',#214049,#27338);
#22112=LINE('',#214053,#27339);
#22113=LINE('',#214142,#27340);
#22114=LINE('',#214146,#27341);
#22115=LINE('',#214235,#27342);
#22116=LINE('',#214239,#27343);
#22117=LINE('',#214328,#27344);
#22118=LINE('',#214332,#27345);
#22119=LINE('',#214421,#27346);
#22120=LINE('',#214425,#27347);
#22121=LINE('',#214514,#27348);
#22122=LINE('',#214518,#27349);
#22123=LINE('',#214607,#27350);
#22124=LINE('',#214611,#27351);
#22125=LINE('',#214700,#27352);
#22126=LINE('',#214704,#27353);
#22127=LINE('',#214790,#27354);
#22128=LINE('',#214794,#27355);
#22129=LINE('',#214883,#27356);
#22130=LINE('',#214887,#27357);
#22131=LINE('',#214976,#27358);
#22132=LINE('',#214980,#27359);
#22133=LINE('',#215069,#27360);
#22134=LINE('',#215073,#27361);
#22135=LINE('',#215162,#27362);
#22136=LINE('',#215166,#27363);
#22137=LINE('',#215255,#27364);
#22138=LINE('',#215259,#27365);
#22139=LINE('',#215348,#27366);
#22140=LINE('',#215352,#27367);
#22141=LINE('',#215441,#27368);
#22142=LINE('',#215445,#27369);
#22143=LINE('',#215534,#27370);
#22144=LINE('',#215538,#27371);
#22145=LINE('',#215627,#27372);
#22146=LINE('',#215631,#27373);
#22147=LINE('',#215720,#27374);
#22148=LINE('',#215724,#27375);
#22149=LINE('',#215813,#27376);
#22150=LINE('',#215817,#27377);
#22151=LINE('',#215906,#27378);
#22152=LINE('',#215910,#27379);
#22153=LINE('',#215999,#27380);
#22154=LINE('',#216003,#27381);
#22155=LINE('',#216092,#27382);
#22156=LINE('',#216096,#27383);
#22157=LINE('',#216177,#27384);
#22158=LINE('',#216181,#27385);
#22159=LINE('',#216264,#27386);
#22160=LINE('',#216268,#27387);
#22161=LINE('',#216351,#27388);
#22162=LINE('',#216355,#27389);
#22163=LINE('',#216438,#27390);
#22164=LINE('',#216442,#27391);
#22165=LINE('',#216525,#27392);
#22166=LINE('',#216529,#27393);
#22167=LINE('',#216612,#27394);
#22168=LINE('',#216616,#27395);
#22169=LINE('',#216699,#27396);
#22170=LINE('',#216703,#27397);
#22171=LINE('',#216786,#27398);
#22172=LINE('',#216790,#27399);
#22173=LINE('',#216873,#27400);
#22174=LINE('',#216877,#27401);
#22175=LINE('',#216960,#27402);
#22176=LINE('',#216964,#27403);
#22177=LINE('',#217047,#27404);
#22178=LINE('',#217051,#27405);
#22179=LINE('',#217134,#27406);
#22180=LINE('',#217138,#27407);
#22181=LINE('',#217221,#27408);
#22182=LINE('',#217225,#27409);
#22183=LINE('',#217308,#27410);
#22184=LINE('',#217312,#27411);
#22185=LINE('',#217395,#27412);
#22186=LINE('',#217399,#27413);
#22187=LINE('',#217482,#27414);
#22188=LINE('',#217486,#27415);
#22189=LINE('',#217569,#27416);
#22190=LINE('',#217573,#27417);
#22191=LINE('',#217656,#27418);
#22192=LINE('',#217660,#27419);
#22193=LINE('',#217743,#27420);
#22194=LINE('',#217747,#27421);
#22195=LINE('',#217830,#27422);
#22196=LINE('',#217834,#27423);
#22197=LINE('',#217917,#27424);
#22198=LINE('',#217921,#27425);
#22199=LINE('',#218004,#27426);
#22200=LINE('',#218008,#27427);
#22201=LINE('',#218091,#27428);
#22202=LINE('',#218095,#27429);
#22203=LINE('',#218178,#27430);
#22204=LINE('',#218182,#27431);
#22205=LINE('',#218265,#27432);
#22206=LINE('',#218269,#27433);
#22207=LINE('',#218352,#27434);
#22208=LINE('',#218356,#27435);
#22209=LINE('',#218439,#27436);
#22210=LINE('',#218443,#27437);
#22211=LINE('',#218526,#27438);
#22212=LINE('',#218530,#27439);
#22213=LINE('',#218613,#27440);
#22214=LINE('',#218617,#27441);
#22215=LINE('',#218700,#27442);
#22216=LINE('',#218704,#27443);
#22217=LINE('',#218748,#27444);
#22218=LINE('',#218790,#27445);
#22219=LINE('',#218794,#27446);
#22220=LINE('',#218877,#27447);
#22221=LINE('',#218881,#27448);
#22222=LINE('',#218964,#27449);
#22223=LINE('',#218968,#27450);
#22224=LINE('',#219051,#27451);
#22225=LINE('',#219055,#27452);
#22226=LINE('',#219138,#27453);
#22227=LINE('',#219142,#27454);
#22228=LINE('',#219225,#27455);
#22229=LINE('',#219229,#27456);
#22230=LINE('',#219312,#27457);
#22231=LINE('',#219316,#27458);
#22232=LINE('',#219399,#27459);
#22233=LINE('',#219403,#27460);
#22234=LINE('',#219486,#27461);
#22235=LINE('',#219490,#27462);
#22236=LINE('',#219573,#27463);
#22237=LINE('',#219577,#27464);
#22238=LINE('',#219660,#27465);
#22239=LINE('',#219664,#27466);
#22240=LINE('',#219747,#27467);
#22241=LINE('',#219751,#27468);
#22242=LINE('',#219834,#27469);
#22243=LINE('',#219838,#27470);
#22244=LINE('',#219921,#27471);
#22245=LINE('',#219925,#27472);
#22246=LINE('',#220008,#27473);
#22247=LINE('',#220012,#27474);
#22248=LINE('',#220092,#27475);
#22249=LINE('',#220096,#27476);
#22250=LINE('',#220179,#27477);
#22251=LINE('',#220183,#27478);
#22252=LINE('',#220266,#27479);
#22253=LINE('',#220270,#27480);
#22254=LINE('',#220353,#27481);
#22255=LINE('',#220357,#27482);
#22256=LINE('',#220440,#27483);
#22257=LINE('',#220444,#27484);
#22258=LINE('',#220527,#27485);
#22259=LINE('',#220531,#27486);
#22260=LINE('',#220614,#27487);
#22261=LINE('',#220618,#27488);
#22262=LINE('',#220701,#27489);
#22263=LINE('',#220705,#27490);
#22264=LINE('',#220788,#27491);
#22265=LINE('',#220792,#27492);
#22266=LINE('',#220875,#27493);
#22267=LINE('',#220879,#27494);
#22268=LINE('',#220962,#27495);
#22269=LINE('',#220966,#27496);
#22270=LINE('',#221049,#27497);
#22271=LINE('',#221053,#27498);
#22272=LINE('',#221136,#27499);
#22273=LINE('',#221140,#27500);
#22274=LINE('',#221223,#27501);
#22275=LINE('',#221227,#27502);
#22276=LINE('',#221310,#27503);
#22277=LINE('',#221314,#27504);
#22278=LINE('',#221359,#27505);
#22279=LINE('',#221363,#27506);
#22280=LINE('',#221370,#27507);
#22281=LINE('',#221374,#27508);
#22282=LINE('',#221382,#27509);
#22283=LINE('',#221383,#27510);
#22284=LINE('',#221389,#27511);
#22285=LINE('',#221392,#27512);
#22286=LINE('',#221398,#27513);
#22287=LINE('',#221402,#27514);
#22288=LINE('',#221410,#27515);
#22289=LINE('',#221411,#27516);
#22290=LINE('',#221429,#27517);
#22291=LINE('',#221436,#27518);
#22292=LINE('',#221439,#27519);
#22293=LINE('',#221442,#27520);
#22294=LINE('',#221448,#27521);
#22295=LINE('',#221451,#27522);
#22296=LINE('',#221457,#27523);
#22297=LINE('',#221464,#27524);
#22298=LINE('',#221467,#27525);
#22299=LINE('',#221470,#27526);
#22300=LINE('',#221488,#27527);
#22301=LINE('',#221495,#27528);
#22302=LINE('',#221498,#27529);
#22303=LINE('',#221501,#27530);
#22304=LINE('',#221507,#27531);
#22305=LINE('',#221510,#27532);
#22306=LINE('',#221516,#27533);
#22307=LINE('',#221523,#27534);
#22308=LINE('',#221526,#27535);
#22309=LINE('',#221529,#27536);
#22310=LINE('',#221547,#27537);
#22311=LINE('',#221554,#27538);
#22312=LINE('',#221557,#27539);
#22313=LINE('',#221560,#27540);
#22314=LINE('',#221566,#27541);
#22315=LINE('',#221569,#27542);
#22316=LINE('',#221575,#27543);
#22317=LINE('',#221582,#27544);
#22318=LINE('',#221585,#27545);
#22319=LINE('',#221588,#27546);
#22320=LINE('',#221606,#27547);
#22321=LINE('',#221613,#27548);
#22322=LINE('',#221616,#27549);
#22323=LINE('',#221619,#27550);
#22324=LINE('',#221625,#27551);
#22325=LINE('',#221628,#27552);
#22326=LINE('',#221634,#27553);
#22327=LINE('',#221641,#27554);
#22328=LINE('',#221644,#27555);
#22329=LINE('',#221647,#27556);
#22330=LINE('',#221665,#27557);
#22331=LINE('',#221672,#27558);
#22332=LINE('',#221675,#27559);
#22333=LINE('',#221678,#27560);
#22334=LINE('',#221684,#27561);
#22335=LINE('',#221687,#27562);
#22336=LINE('',#221693,#27563);
#22337=LINE('',#221700,#27564);
#22338=LINE('',#221703,#27565);
#22339=LINE('',#221706,#27566);
#22340=LINE('',#221724,#27567);
#22341=LINE('',#221731,#27568);
#22342=LINE('',#221734,#27569);
#22343=LINE('',#221737,#27570);
#22344=LINE('',#221743,#27571);
#22345=LINE('',#221746,#27572);
#22346=LINE('',#221752,#27573);
#22347=LINE('',#221759,#27574);
#22348=LINE('',#221762,#27575);
#22349=LINE('',#221765,#27576);
#22350=LINE('',#221783,#27577);
#22351=LINE('',#221790,#27578);
#22352=LINE('',#221793,#27579);
#22353=LINE('',#221796,#27580);
#22354=LINE('',#221802,#27581);
#22355=LINE('',#221805,#27582);
#22356=LINE('',#221811,#27583);
#22357=LINE('',#221818,#27584);
#22358=LINE('',#221821,#27585);
#22359=LINE('',#221824,#27586);
#22360=LINE('',#221842,#27587);
#22361=LINE('',#221849,#27588);
#22362=LINE('',#221852,#27589);
#22363=LINE('',#221855,#27590);
#22364=LINE('',#221861,#27591);
#22365=LINE('',#221864,#27592);
#22366=LINE('',#221870,#27593);
#22367=LINE('',#221877,#27594);
#22368=LINE('',#221880,#27595);
#22369=LINE('',#221883,#27596);
#22370=LINE('',#221901,#27597);
#22371=LINE('',#221908,#27598);
#22372=LINE('',#221911,#27599);
#22373=LINE('',#221914,#27600);
#22374=LINE('',#221920,#27601);
#22375=LINE('',#221923,#27602);
#22376=LINE('',#221929,#27603);
#22377=LINE('',#221936,#27604);
#22378=LINE('',#221939,#27605);
#22379=LINE('',#221942,#27606);
#22380=LINE('',#221960,#27607);
#22381=LINE('',#221967,#27608);
#22382=LINE('',#221970,#27609);
#22383=LINE('',#221973,#27610);
#22384=LINE('',#221979,#27611);
#22385=LINE('',#221982,#27612);
#22386=LINE('',#221988,#27613);
#22387=LINE('',#221995,#27614);
#22388=LINE('',#221998,#27615);
#22389=LINE('',#222001,#27616);
#22390=LINE('',#222019,#27617);
#22391=LINE('',#222026,#27618);
#22392=LINE('',#222029,#27619);
#22393=LINE('',#222032,#27620);
#22394=LINE('',#222038,#27621);
#22395=LINE('',#222041,#27622);
#22396=LINE('',#222047,#27623);
#22397=LINE('',#222054,#27624);
#22398=LINE('',#222057,#27625);
#22399=LINE('',#222060,#27626);
#22400=LINE('',#222078,#27627);
#22401=LINE('',#222085,#27628);
#22402=LINE('',#222088,#27629);
#22403=LINE('',#222091,#27630);
#22404=LINE('',#222097,#27631);
#22405=LINE('',#222100,#27632);
#22406=LINE('',#222106,#27633);
#22407=LINE('',#222113,#27634);
#22408=LINE('',#222116,#27635);
#22409=LINE('',#222119,#27636);
#22410=LINE('',#222137,#27637);
#22411=LINE('',#222144,#27638);
#22412=LINE('',#222147,#27639);
#22413=LINE('',#222150,#27640);
#22414=LINE('',#222156,#27641);
#22415=LINE('',#222159,#27642);
#22416=LINE('',#222165,#27643);
#22417=LINE('',#222172,#27644);
#22418=LINE('',#222175,#27645);
#22419=LINE('',#222178,#27646);
#22420=LINE('',#222196,#27647);
#22421=LINE('',#222203,#27648);
#22422=LINE('',#222206,#27649);
#22423=LINE('',#222209,#27650);
#22424=LINE('',#222215,#27651);
#22425=LINE('',#222218,#27652);
#22426=LINE('',#222224,#27653);
#22427=LINE('',#222231,#27654);
#22428=LINE('',#222234,#27655);
#22429=LINE('',#222237,#27656);
#22430=LINE('',#222255,#27657);
#22431=LINE('',#222262,#27658);
#22432=LINE('',#222265,#27659);
#22433=LINE('',#222268,#27660);
#22434=LINE('',#222274,#27661);
#22435=LINE('',#222277,#27662);
#22436=LINE('',#222283,#27663);
#22437=LINE('',#222290,#27664);
#22438=LINE('',#222293,#27665);
#22439=LINE('',#222296,#27666);
#22440=LINE('',#222314,#27667);
#22441=LINE('',#222321,#27668);
#22442=LINE('',#222324,#27669);
#22443=LINE('',#222327,#27670);
#22444=LINE('',#222333,#27671);
#22445=LINE('',#222336,#27672);
#22446=LINE('',#222342,#27673);
#22447=LINE('',#222349,#27674);
#22448=LINE('',#222352,#27675);
#22449=LINE('',#222355,#27676);
#22450=LINE('',#222373,#27677);
#22451=LINE('',#222380,#27678);
#22452=LINE('',#222383,#27679);
#22453=LINE('',#222386,#27680);
#22454=LINE('',#222392,#27681);
#22455=LINE('',#222395,#27682);
#22456=LINE('',#222401,#27683);
#22457=LINE('',#222408,#27684);
#22458=LINE('',#222411,#27685);
#22459=LINE('',#222414,#27686);
#22460=LINE('',#222432,#27687);
#22461=LINE('',#222439,#27688);
#22462=LINE('',#222442,#27689);
#22463=LINE('',#222445,#27690);
#22464=LINE('',#222451,#27691);
#22465=LINE('',#222454,#27692);
#22466=LINE('',#222460,#27693);
#22467=LINE('',#222467,#27694);
#22468=LINE('',#222470,#27695);
#22469=LINE('',#222473,#27696);
#22470=LINE('',#222491,#27697);
#22471=LINE('',#222498,#27698);
#22472=LINE('',#222501,#27699);
#22473=LINE('',#222504,#27700);
#22474=LINE('',#222510,#27701);
#22475=LINE('',#222513,#27702);
#22476=LINE('',#222519,#27703);
#22477=LINE('',#222526,#27704);
#22478=LINE('',#222529,#27705);
#22479=LINE('',#222532,#27706);
#22480=LINE('',#222550,#27707);
#22481=LINE('',#222557,#27708);
#22482=LINE('',#222560,#27709);
#22483=LINE('',#222563,#27710);
#22484=LINE('',#222569,#27711);
#22485=LINE('',#222572,#27712);
#22486=LINE('',#222578,#27713);
#22487=LINE('',#222585,#27714);
#22488=LINE('',#222588,#27715);
#22489=LINE('',#222591,#27716);
#22490=LINE('',#222609,#27717);
#22491=LINE('',#222616,#27718);
#22492=LINE('',#222619,#27719);
#22493=LINE('',#222622,#27720);
#22494=LINE('',#222628,#27721);
#22495=LINE('',#222631,#27722);
#22496=LINE('',#222637,#27723);
#22497=LINE('',#222644,#27724);
#22498=LINE('',#222647,#27725);
#22499=LINE('',#222650,#27726);
#22500=LINE('',#222668,#27727);
#22501=LINE('',#222675,#27728);
#22502=LINE('',#222678,#27729);
#22503=LINE('',#222681,#27730);
#22504=LINE('',#222687,#27731);
#22505=LINE('',#222690,#27732);
#22506=LINE('',#222696,#27733);
#22507=LINE('',#222703,#27734);
#22508=LINE('',#222706,#27735);
#22509=LINE('',#222709,#27736);
#22510=LINE('',#222727,#27737);
#22511=LINE('',#222734,#27738);
#22512=LINE('',#222737,#27739);
#22513=LINE('',#222740,#27740);
#22514=LINE('',#222746,#27741);
#22515=LINE('',#222749,#27742);
#22516=LINE('',#222755,#27743);
#22517=LINE('',#222762,#27744);
#22518=LINE('',#222765,#27745);
#22519=LINE('',#222768,#27746);
#22520=LINE('',#222786,#27747);
#22521=LINE('',#222793,#27748);
#22522=LINE('',#222796,#27749);
#22523=LINE('',#222799,#27750);
#22524=LINE('',#222805,#27751);
#22525=LINE('',#222808,#27752);
#22526=LINE('',#222814,#27753);
#22527=LINE('',#222821,#27754);
#22528=LINE('',#222824,#27755);
#22529=LINE('',#222827,#27756);
#22530=LINE('',#222845,#27757);
#22531=LINE('',#222852,#27758);
#22532=LINE('',#222855,#27759);
#22533=LINE('',#222858,#27760);
#22534=LINE('',#222864,#27761);
#22535=LINE('',#222867,#27762);
#22536=LINE('',#222873,#27763);
#22537=LINE('',#222880,#27764);
#22538=LINE('',#222883,#27765);
#22539=LINE('',#222886,#27766);
#22540=LINE('',#222904,#27767);
#22541=LINE('',#222911,#27768);
#22542=LINE('',#222914,#27769);
#22543=LINE('',#222917,#27770);
#22544=LINE('',#222923,#27771);
#22545=LINE('',#222926,#27772);
#22546=LINE('',#222932,#27773);
#22547=LINE('',#222939,#27774);
#22548=LINE('',#222942,#27775);
#22549=LINE('',#222945,#27776);
#22550=LINE('',#222963,#27777);
#22551=LINE('',#222970,#27778);
#22552=LINE('',#222973,#27779);
#22553=LINE('',#222976,#27780);
#22554=LINE('',#222982,#27781);
#22555=LINE('',#222985,#27782);
#22556=LINE('',#222991,#27783);
#22557=LINE('',#222998,#27784);
#22558=LINE('',#223001,#27785);
#22559=LINE('',#223004,#27786);
#22560=LINE('',#223022,#27787);
#22561=LINE('',#223029,#27788);
#22562=LINE('',#223032,#27789);
#22563=LINE('',#223035,#27790);
#22564=LINE('',#223041,#27791);
#22565=LINE('',#223044,#27792);
#22566=LINE('',#223050,#27793);
#22567=LINE('',#223057,#27794);
#22568=LINE('',#223060,#27795);
#22569=LINE('',#223063,#27796);
#22570=LINE('',#223081,#27797);
#22571=LINE('',#223088,#27798);
#22572=LINE('',#223091,#27799);
#22573=LINE('',#223094,#27800);
#22574=LINE('',#223100,#27801);
#22575=LINE('',#223103,#27802);
#22576=LINE('',#223109,#27803);
#22577=LINE('',#223116,#27804);
#22578=LINE('',#223119,#27805);
#22579=LINE('',#223122,#27806);
#22580=LINE('',#223140,#27807);
#22581=LINE('',#223147,#27808);
#22582=LINE('',#223150,#27809);
#22583=LINE('',#223153,#27810);
#22584=LINE('',#223159,#27811);
#22585=LINE('',#223162,#27812);
#22586=LINE('',#223168,#27813);
#22587=LINE('',#223175,#27814);
#22588=LINE('',#223178,#27815);
#22589=LINE('',#223181,#27816);
#22590=LINE('',#223199,#27817);
#22591=LINE('',#223206,#27818);
#22592=LINE('',#223209,#27819);
#22593=LINE('',#223212,#27820);
#22594=LINE('',#223218,#27821);
#22595=LINE('',#223221,#27822);
#22596=LINE('',#223227,#27823);
#22597=LINE('',#223234,#27824);
#22598=LINE('',#223237,#27825);
#22599=LINE('',#223240,#27826);
#22600=LINE('',#223258,#27827);
#22601=LINE('',#223265,#27828);
#22602=LINE('',#223268,#27829);
#22603=LINE('',#223271,#27830);
#22604=LINE('',#223277,#27831);
#22605=LINE('',#223280,#27832);
#22606=LINE('',#223286,#27833);
#22607=LINE('',#223293,#27834);
#22608=LINE('',#223296,#27835);
#22609=LINE('',#223299,#27836);
#22610=LINE('',#223317,#27837);
#22611=LINE('',#223324,#27838);
#22612=LINE('',#223327,#27839);
#22613=LINE('',#223330,#27840);
#22614=LINE('',#223336,#27841);
#22615=LINE('',#223339,#27842);
#22616=LINE('',#223345,#27843);
#22617=LINE('',#223352,#27844);
#22618=LINE('',#223355,#27845);
#22619=LINE('',#223358,#27846);
#22620=LINE('',#223376,#27847);
#22621=LINE('',#223383,#27848);
#22622=LINE('',#223386,#27849);
#22623=LINE('',#223389,#27850);
#22624=LINE('',#223395,#27851);
#22625=LINE('',#223398,#27852);
#22626=LINE('',#223404,#27853);
#22627=LINE('',#223411,#27854);
#22628=LINE('',#223414,#27855);
#22629=LINE('',#223417,#27856);
#22630=LINE('',#223435,#27857);
#22631=LINE('',#223442,#27858);
#22632=LINE('',#223445,#27859);
#22633=LINE('',#223448,#27860);
#22634=LINE('',#223454,#27861);
#22635=LINE('',#223457,#27862);
#22636=LINE('',#223463,#27863);
#22637=LINE('',#223470,#27864);
#22638=LINE('',#223473,#27865);
#22639=LINE('',#223476,#27866);
#22640=LINE('',#223494,#27867);
#22641=LINE('',#223501,#27868);
#22642=LINE('',#223504,#27869);
#22643=LINE('',#223507,#27870);
#22644=LINE('',#223513,#27871);
#22645=LINE('',#223516,#27872);
#22646=LINE('',#223522,#27873);
#22647=LINE('',#223529,#27874);
#22648=LINE('',#223532,#27875);
#22649=LINE('',#223535,#27876);
#22650=LINE('',#223553,#27877);
#22651=LINE('',#223560,#27878);
#22652=LINE('',#223563,#27879);
#22653=LINE('',#223566,#27880);
#22654=LINE('',#223572,#27881);
#22655=LINE('',#223575,#27882);
#22656=LINE('',#223581,#27883);
#22657=LINE('',#223588,#27884);
#22658=LINE('',#223591,#27885);
#22659=LINE('',#223594,#27886);
#22660=LINE('',#223612,#27887);
#22661=LINE('',#223619,#27888);
#22662=LINE('',#223622,#27889);
#22663=LINE('',#223625,#27890);
#22664=LINE('',#223631,#27891);
#22665=LINE('',#223634,#27892);
#22666=LINE('',#223640,#27893);
#22667=LINE('',#223647,#27894);
#22668=LINE('',#223650,#27895);
#22669=LINE('',#223653,#27896);
#22670=LINE('',#223671,#27897);
#22671=LINE('',#223678,#27898);
#22672=LINE('',#223681,#27899);
#22673=LINE('',#223684,#27900);
#22674=LINE('',#223690,#27901);
#22675=LINE('',#223693,#27902);
#22676=LINE('',#223699,#27903);
#22677=LINE('',#223706,#27904);
#22678=LINE('',#223709,#27905);
#22679=LINE('',#223712,#27906);
#22680=LINE('',#223730,#27907);
#22681=LINE('',#223737,#27908);
#22682=LINE('',#223740,#27909);
#22683=LINE('',#223743,#27910);
#22684=LINE('',#223749,#27911);
#22685=LINE('',#223752,#27912);
#22686=LINE('',#223758,#27913);
#22687=LINE('',#223765,#27914);
#22688=LINE('',#223768,#27915);
#22689=LINE('',#223771,#27916);
#22690=LINE('',#223789,#27917);
#22691=LINE('',#223796,#27918);
#22692=LINE('',#223799,#27919);
#22693=LINE('',#223802,#27920);
#22694=LINE('',#223808,#27921);
#22695=LINE('',#223811,#27922);
#22696=LINE('',#223817,#27923);
#22697=LINE('',#223824,#27924);
#22698=LINE('',#223827,#27925);
#22699=LINE('',#223830,#27926);
#22700=LINE('',#223848,#27927);
#22701=LINE('',#223855,#27928);
#22702=LINE('',#223858,#27929);
#22703=LINE('',#223861,#27930);
#22704=LINE('',#223867,#27931);
#22705=LINE('',#223870,#27932);
#22706=LINE('',#223876,#27933);
#22707=LINE('',#223883,#27934);
#22708=LINE('',#223886,#27935);
#22709=LINE('',#223889,#27936);
#22710=LINE('',#223907,#27937);
#22711=LINE('',#223914,#27938);
#22712=LINE('',#223917,#27939);
#22713=LINE('',#223920,#27940);
#22714=LINE('',#223926,#27941);
#22715=LINE('',#223929,#27942);
#22716=LINE('',#223935,#27943);
#22717=LINE('',#223942,#27944);
#22718=LINE('',#223945,#27945);
#22719=LINE('',#223948,#27946);
#22720=LINE('',#223966,#27947);
#22721=LINE('',#223973,#27948);
#22722=LINE('',#223976,#27949);
#22723=LINE('',#223979,#27950);
#22724=LINE('',#223985,#27951);
#22725=LINE('',#223988,#27952);
#22726=LINE('',#223994,#27953);
#22727=LINE('',#224001,#27954);
#22728=LINE('',#224004,#27955);
#22729=LINE('',#224007,#27956);
#22730=LINE('',#224025,#27957);
#22731=LINE('',#224032,#27958);
#22732=LINE('',#224035,#27959);
#22733=LINE('',#224038,#27960);
#22734=LINE('',#224044,#27961);
#22735=LINE('',#224047,#27962);
#22736=LINE('',#224053,#27963);
#22737=LINE('',#224060,#27964);
#22738=LINE('',#224063,#27965);
#22739=LINE('',#224066,#27966);
#22740=LINE('',#224084,#27967);
#22741=LINE('',#224091,#27968);
#22742=LINE('',#224094,#27969);
#22743=LINE('',#224097,#27970);
#22744=LINE('',#224103,#27971);
#22745=LINE('',#224106,#27972);
#22746=LINE('',#224112,#27973);
#22747=LINE('',#224119,#27974);
#22748=LINE('',#224122,#27975);
#22749=LINE('',#224125,#27976);
#22750=LINE('',#224143,#27977);
#22751=LINE('',#224150,#27978);
#22752=LINE('',#224153,#27979);
#22753=LINE('',#224156,#27980);
#22754=LINE('',#224162,#27981);
#22755=LINE('',#224165,#27982);
#22756=LINE('',#224171,#27983);
#22757=LINE('',#224178,#27984);
#22758=LINE('',#224181,#27985);
#22759=LINE('',#224184,#27986);
#22760=LINE('',#224202,#27987);
#22761=LINE('',#224209,#27988);
#22762=LINE('',#224212,#27989);
#22763=LINE('',#224215,#27990);
#22764=LINE('',#224221,#27991);
#22765=LINE('',#224224,#27992);
#22766=LINE('',#224230,#27993);
#22767=LINE('',#224237,#27994);
#22768=LINE('',#224240,#27995);
#22769=LINE('',#224243,#27996);
#22770=LINE('',#224261,#27997);
#22771=LINE('',#224268,#27998);
#22772=LINE('',#224271,#27999);
#22773=LINE('',#224274,#28000);
#22774=LINE('',#224280,#28001);
#22775=LINE('',#224283,#28002);
#22776=LINE('',#224289,#28003);
#22777=LINE('',#224296,#28004);
#22778=LINE('',#224299,#28005);
#22779=LINE('',#224302,#28006);
#22780=LINE('',#224320,#28007);
#22781=LINE('',#224327,#28008);
#22782=LINE('',#224330,#28009);
#22783=LINE('',#224333,#28010);
#22784=LINE('',#224339,#28011);
#22785=LINE('',#224342,#28012);
#22786=LINE('',#224348,#28013);
#22787=LINE('',#224355,#28014);
#22788=LINE('',#224358,#28015);
#22789=LINE('',#224361,#28016);
#22790=LINE('',#224379,#28017);
#22791=LINE('',#224386,#28018);
#22792=LINE('',#224389,#28019);
#22793=LINE('',#224392,#28020);
#22794=LINE('',#224398,#28021);
#22795=LINE('',#224401,#28022);
#22796=LINE('',#224407,#28023);
#22797=LINE('',#224414,#28024);
#22798=LINE('',#224417,#28025);
#22799=LINE('',#224420,#28026);
#22800=LINE('',#224438,#28027);
#22801=LINE('',#224445,#28028);
#22802=LINE('',#224448,#28029);
#22803=LINE('',#224451,#28030);
#22804=LINE('',#224457,#28031);
#22805=LINE('',#224460,#28032);
#22806=LINE('',#224466,#28033);
#22807=LINE('',#224473,#28034);
#22808=LINE('',#224476,#28035);
#22809=LINE('',#224479,#28036);
#22810=LINE('',#224497,#28037);
#22811=LINE('',#224504,#28038);
#22812=LINE('',#224507,#28039);
#22813=LINE('',#224510,#28040);
#22814=LINE('',#224516,#28041);
#22815=LINE('',#224519,#28042);
#22816=LINE('',#224525,#28043);
#22817=LINE('',#224532,#28044);
#22818=LINE('',#224535,#28045);
#22819=LINE('',#224538,#28046);
#22820=LINE('',#224556,#28047);
#22821=LINE('',#224563,#28048);
#22822=LINE('',#224566,#28049);
#22823=LINE('',#224569,#28050);
#22824=LINE('',#224575,#28051);
#22825=LINE('',#224578,#28052);
#22826=LINE('',#224584,#28053);
#22827=LINE('',#224591,#28054);
#22828=LINE('',#224594,#28055);
#22829=LINE('',#224597,#28056);
#22830=LINE('',#224615,#28057);
#22831=LINE('',#224622,#28058);
#22832=LINE('',#224625,#28059);
#22833=LINE('',#224628,#28060);
#22834=LINE('',#224634,#28061);
#22835=LINE('',#224637,#28062);
#22836=LINE('',#224643,#28063);
#22837=LINE('',#224650,#28064);
#22838=LINE('',#224653,#28065);
#22839=LINE('',#224656,#28066);
#22840=LINE('',#224674,#28067);
#22841=LINE('',#224681,#28068);
#22842=LINE('',#224684,#28069);
#22843=LINE('',#224687,#28070);
#22844=LINE('',#224693,#28071);
#22845=LINE('',#224696,#28072);
#22846=LINE('',#224702,#28073);
#22847=LINE('',#224709,#28074);
#22848=LINE('',#224712,#28075);
#22849=LINE('',#224715,#28076);
#22850=LINE('',#224733,#28077);
#22851=LINE('',#224740,#28078);
#22852=LINE('',#224743,#28079);
#22853=LINE('',#224746,#28080);
#22854=LINE('',#224752,#28081);
#22855=LINE('',#224755,#28082);
#22856=LINE('',#224761,#28083);
#22857=LINE('',#224768,#28084);
#22858=LINE('',#224771,#28085);
#22859=LINE('',#224774,#28086);
#22860=LINE('',#224792,#28087);
#22861=LINE('',#224799,#28088);
#22862=LINE('',#224802,#28089);
#22863=LINE('',#224805,#28090);
#22864=LINE('',#224811,#28091);
#22865=LINE('',#224814,#28092);
#22866=LINE('',#224820,#28093);
#22867=LINE('',#224827,#28094);
#22868=LINE('',#224830,#28095);
#22869=LINE('',#224833,#28096);
#22870=LINE('',#224852,#28097);
#22871=LINE('',#224859,#28098);
#22872=LINE('',#224862,#28099);
#22873=LINE('',#224865,#28100);
#22874=LINE('',#224871,#28101);
#22875=LINE('',#224874,#28102);
#22876=LINE('',#224880,#28103);
#22877=LINE('',#224887,#28104);
#22878=LINE('',#224890,#28105);
#22879=LINE('',#224893,#28106);
#22880=LINE('',#224911,#28107);
#22881=LINE('',#224915,#28108);
#22882=LINE('',#224922,#28109);
#22883=LINE('',#224924,#28110);
#22884=LINE('',#224926,#28111);
#22885=LINE('',#224930,#28112);
#22886=LINE('',#224932,#28113);
#22887=LINE('',#224936,#28114);
#22888=LINE('',#224940,#28115);
#22889=LINE('',#224941,#28116);
#22890=LINE('',#224947,#28117);
#22891=LINE('',#224949,#28118);
#22892=LINE('',#224951,#28119);
#22893=LINE('',#224955,#28120);
#22894=LINE('',#224957,#28121);
#22895=LINE('',#224961,#28122);
#22896=LINE('',#224965,#28123);
#22897=LINE('',#224966,#28124);
#22898=LINE('',#225386,#28125);
#22899=LINE('',#225390,#28126);
#22900=LINE('',#225397,#28127);
#22901=LINE('',#225399,#28128);
#22902=LINE('',#225401,#28129);
#22903=LINE('',#225405,#28130);
#22904=LINE('',#225407,#28131);
#22905=LINE('',#225411,#28132);
#22906=LINE('',#225415,#28133);
#22907=LINE('',#225416,#28134);
#22908=LINE('',#225422,#28135);
#22909=LINE('',#225424,#28136);
#22910=LINE('',#225426,#28137);
#22911=LINE('',#225430,#28138);
#22912=LINE('',#225432,#28139);
#22913=LINE('',#225436,#28140);
#22914=LINE('',#225440,#28141);
#22915=LINE('',#225441,#28142);
#22916=LINE('',#225445,#28143);
#22917=LINE('',#225449,#28144);
#22918=LINE('',#225456,#28145);
#22919=LINE('',#225458,#28146);
#22920=LINE('',#225460,#28147);
#22921=LINE('',#225464,#28148);
#22922=LINE('',#225466,#28149);
#22923=LINE('',#225470,#28150);
#22924=LINE('',#225474,#28151);
#22925=LINE('',#225475,#28152);
#22926=LINE('',#225481,#28153);
#22927=LINE('',#225483,#28154);
#22928=LINE('',#225485,#28155);
#22929=LINE('',#225489,#28156);
#22930=LINE('',#225491,#28157);
#22931=LINE('',#225495,#28158);
#22932=LINE('',#225499,#28159);
#22933=LINE('',#225500,#28160);
#22934=LINE('',#225504,#28161);
#22935=LINE('',#225508,#28162);
#22936=LINE('',#225515,#28163);
#22937=LINE('',#225517,#28164);
#22938=LINE('',#225519,#28165);
#22939=LINE('',#225523,#28166);
#22940=LINE('',#225525,#28167);
#22941=LINE('',#225529,#28168);
#22942=LINE('',#225533,#28169);
#22943=LINE('',#225534,#28170);
#22944=LINE('',#225540,#28171);
#22945=LINE('',#225542,#28172);
#22946=LINE('',#225544,#28173);
#22947=LINE('',#225548,#28174);
#22948=LINE('',#225550,#28175);
#22949=LINE('',#225554,#28176);
#22950=LINE('',#225558,#28177);
#22951=LINE('',#225559,#28178);
#22952=LINE('',#225563,#28179);
#22953=LINE('',#225567,#28180);
#22954=LINE('',#225574,#28181);
#22955=LINE('',#225576,#28182);
#22956=LINE('',#225578,#28183);
#22957=LINE('',#225582,#28184);
#22958=LINE('',#225584,#28185);
#22959=LINE('',#225588,#28186);
#22960=LINE('',#225592,#28187);
#22961=LINE('',#225593,#28188);
#22962=LINE('',#225599,#28189);
#22963=LINE('',#225601,#28190);
#22964=LINE('',#225603,#28191);
#22965=LINE('',#225607,#28192);
#22966=LINE('',#225609,#28193);
#22967=LINE('',#225613,#28194);
#22968=LINE('',#225617,#28195);
#22969=LINE('',#225618,#28196);
#22970=LINE('',#225622,#28197);
#22971=LINE('',#225626,#28198);
#22972=LINE('',#225633,#28199);
#22973=LINE('',#225635,#28200);
#22974=LINE('',#225637,#28201);
#22975=LINE('',#225641,#28202);
#22976=LINE('',#225643,#28203);
#22977=LINE('',#225647,#28204);
#22978=LINE('',#225651,#28205);
#22979=LINE('',#225652,#28206);
#22980=LINE('',#225658,#28207);
#22981=LINE('',#225660,#28208);
#22982=LINE('',#225662,#28209);
#22983=LINE('',#225666,#28210);
#22984=LINE('',#225668,#28211);
#22985=LINE('',#225672,#28212);
#22986=LINE('',#225676,#28213);
#22987=LINE('',#225677,#28214);
#22988=LINE('',#225681,#28215);
#22989=LINE('',#225685,#28216);
#22990=LINE('',#225692,#28217);
#22991=LINE('',#225694,#28218);
#22992=LINE('',#225696,#28219);
#22993=LINE('',#225700,#28220);
#22994=LINE('',#225702,#28221);
#22995=LINE('',#225706,#28222);
#22996=LINE('',#225710,#28223);
#22997=LINE('',#225711,#28224);
#22998=LINE('',#225717,#28225);
#22999=LINE('',#225719,#28226);
#23000=LINE('',#225721,#28227);
#23001=LINE('',#225725,#28228);
#23002=LINE('',#225727,#28229);
#23003=LINE('',#225731,#28230);
#23004=LINE('',#225735,#28231);
#23005=LINE('',#225736,#28232);
#23006=LINE('',#225740,#28233);
#23007=LINE('',#225744,#28234);
#23008=LINE('',#225751,#28235);
#23009=LINE('',#225753,#28236);
#23010=LINE('',#225755,#28237);
#23011=LINE('',#225759,#28238);
#23012=LINE('',#225761,#28239);
#23013=LINE('',#225765,#28240);
#23014=LINE('',#225769,#28241);
#23015=LINE('',#225770,#28242);
#23016=LINE('',#225776,#28243);
#23017=LINE('',#225778,#28244);
#23018=LINE('',#225780,#28245);
#23019=LINE('',#225784,#28246);
#23020=LINE('',#225786,#28247);
#23021=LINE('',#225790,#28248);
#23022=LINE('',#225794,#28249);
#23023=LINE('',#225795,#28250);
#23024=LINE('',#225799,#28251);
#23025=LINE('',#225803,#28252);
#23026=LINE('',#225810,#28253);
#23027=LINE('',#225812,#28254);
#23028=LINE('',#225814,#28255);
#23029=LINE('',#225818,#28256);
#23030=LINE('',#225820,#28257);
#23031=LINE('',#225824,#28258);
#23032=LINE('',#225828,#28259);
#23033=LINE('',#225829,#28260);
#23034=LINE('',#225835,#28261);
#23035=LINE('',#225837,#28262);
#23036=LINE('',#225839,#28263);
#23037=LINE('',#225843,#28264);
#23038=LINE('',#225845,#28265);
#23039=LINE('',#225849,#28266);
#23040=LINE('',#225853,#28267);
#23041=LINE('',#225854,#28268);
#23042=LINE('',#225858,#28269);
#23043=LINE('',#225862,#28270);
#23044=LINE('',#225869,#28271);
#23045=LINE('',#225871,#28272);
#23046=LINE('',#225873,#28273);
#23047=LINE('',#225877,#28274);
#23048=LINE('',#225879,#28275);
#23049=LINE('',#225883,#28276);
#23050=LINE('',#225887,#28277);
#23051=LINE('',#225888,#28278);
#23052=LINE('',#225894,#28279);
#23053=LINE('',#225896,#28280);
#23054=LINE('',#225898,#28281);
#23055=LINE('',#225902,#28282);
#23056=LINE('',#225904,#28283);
#23057=LINE('',#225908,#28284);
#23058=LINE('',#225912,#28285);
#23059=LINE('',#225913,#28286);
#23060=LINE('',#225917,#28287);
#23061=LINE('',#225921,#28288);
#23062=LINE('',#225928,#28289);
#23063=LINE('',#225930,#28290);
#23064=LINE('',#225932,#28291);
#23065=LINE('',#225936,#28292);
#23066=LINE('',#225938,#28293);
#23067=LINE('',#225942,#28294);
#23068=LINE('',#225946,#28295);
#23069=LINE('',#225947,#28296);
#23070=LINE('',#225953,#28297);
#23071=LINE('',#225955,#28298);
#23072=LINE('',#225957,#28299);
#23073=LINE('',#225961,#28300);
#23074=LINE('',#225963,#28301);
#23075=LINE('',#225967,#28302);
#23076=LINE('',#225971,#28303);
#23077=LINE('',#225972,#28304);
#23078=LINE('',#225976,#28305);
#23079=LINE('',#225980,#28306);
#23080=LINE('',#225987,#28307);
#23081=LINE('',#225989,#28308);
#23082=LINE('',#225991,#28309);
#23083=LINE('',#225995,#28310);
#23084=LINE('',#225997,#28311);
#23085=LINE('',#226001,#28312);
#23086=LINE('',#226005,#28313);
#23087=LINE('',#226006,#28314);
#23088=LINE('',#226012,#28315);
#23089=LINE('',#226014,#28316);
#23090=LINE('',#226016,#28317);
#23091=LINE('',#226020,#28318);
#23092=LINE('',#226022,#28319);
#23093=LINE('',#226026,#28320);
#23094=LINE('',#226030,#28321);
#23095=LINE('',#226031,#28322);
#23096=LINE('',#226035,#28323);
#23097=LINE('',#226039,#28324);
#23098=LINE('',#226046,#28325);
#23099=LINE('',#226048,#28326);
#23100=LINE('',#226050,#28327);
#23101=LINE('',#226054,#28328);
#23102=LINE('',#226056,#28329);
#23103=LINE('',#226060,#28330);
#23104=LINE('',#226064,#28331);
#23105=LINE('',#226065,#28332);
#23106=LINE('',#226071,#28333);
#23107=LINE('',#226073,#28334);
#23108=LINE('',#226075,#28335);
#23109=LINE('',#226079,#28336);
#23110=LINE('',#226081,#28337);
#23111=LINE('',#226085,#28338);
#23112=LINE('',#226089,#28339);
#23113=LINE('',#226090,#28340);
#23114=LINE('',#226094,#28341);
#23115=LINE('',#226098,#28342);
#23116=LINE('',#226105,#28343);
#23117=LINE('',#226107,#28344);
#23118=LINE('',#226109,#28345);
#23119=LINE('',#226113,#28346);
#23120=LINE('',#226115,#28347);
#23121=LINE('',#226119,#28348);
#23122=LINE('',#226123,#28349);
#23123=LINE('',#226124,#28350);
#23124=LINE('',#226130,#28351);
#23125=LINE('',#226132,#28352);
#23126=LINE('',#226134,#28353);
#23127=LINE('',#226138,#28354);
#23128=LINE('',#226140,#28355);
#23129=LINE('',#226144,#28356);
#23130=LINE('',#226148,#28357);
#23131=LINE('',#226149,#28358);
#23132=LINE('',#226153,#28359);
#23133=LINE('',#226157,#28360);
#23134=LINE('',#226164,#28361);
#23135=LINE('',#226166,#28362);
#23136=LINE('',#226168,#28363);
#23137=LINE('',#226172,#28364);
#23138=LINE('',#226174,#28365);
#23139=LINE('',#226178,#28366);
#23140=LINE('',#226182,#28367);
#23141=LINE('',#226183,#28368);
#23142=LINE('',#226189,#28369);
#23143=LINE('',#226191,#28370);
#23144=LINE('',#226193,#28371);
#23145=LINE('',#226197,#28372);
#23146=LINE('',#226199,#28373);
#23147=LINE('',#226203,#28374);
#23148=LINE('',#226207,#28375);
#23149=LINE('',#226208,#28376);
#23150=LINE('',#226212,#28377);
#23151=LINE('',#226216,#28378);
#23152=LINE('',#226223,#28379);
#23153=LINE('',#226225,#28380);
#23154=LINE('',#226227,#28381);
#23155=LINE('',#226231,#28382);
#23156=LINE('',#226233,#28383);
#23157=LINE('',#226237,#28384);
#23158=LINE('',#226241,#28385);
#23159=LINE('',#226242,#28386);
#23160=LINE('',#226248,#28387);
#23161=LINE('',#226250,#28388);
#23162=LINE('',#226252,#28389);
#23163=LINE('',#226256,#28390);
#23164=LINE('',#226258,#28391);
#23165=LINE('',#226262,#28392);
#23166=LINE('',#226266,#28393);
#23167=LINE('',#226267,#28394);
#23168=LINE('',#226271,#28395);
#23169=LINE('',#226275,#28396);
#23170=LINE('',#226282,#28397);
#23171=LINE('',#226284,#28398);
#23172=LINE('',#226286,#28399);
#23173=LINE('',#226290,#28400);
#23174=LINE('',#226292,#28401);
#23175=LINE('',#226296,#28402);
#23176=LINE('',#226300,#28403);
#23177=LINE('',#226301,#28404);
#23178=LINE('',#226307,#28405);
#23179=LINE('',#226309,#28406);
#23180=LINE('',#226311,#28407);
#23181=LINE('',#226315,#28408);
#23182=LINE('',#226317,#28409);
#23183=LINE('',#226321,#28410);
#23184=LINE('',#226325,#28411);
#23185=LINE('',#226326,#28412);
#23186=LINE('',#226330,#28413);
#23187=LINE('',#226334,#28414);
#23188=LINE('',#226341,#28415);
#23189=LINE('',#226343,#28416);
#23190=LINE('',#226345,#28417);
#23191=LINE('',#226349,#28418);
#23192=LINE('',#226351,#28419);
#23193=LINE('',#226355,#28420);
#23194=LINE('',#226359,#28421);
#23195=LINE('',#226360,#28422);
#23196=LINE('',#226366,#28423);
#23197=LINE('',#226368,#28424);
#23198=LINE('',#226370,#28425);
#23199=LINE('',#226374,#28426);
#23200=LINE('',#226376,#28427);
#23201=LINE('',#226380,#28428);
#23202=LINE('',#226384,#28429);
#23203=LINE('',#226385,#28430);
#23204=LINE('',#226389,#28431);
#23205=LINE('',#226393,#28432);
#23206=LINE('',#226400,#28433);
#23207=LINE('',#226402,#28434);
#23208=LINE('',#226404,#28435);
#23209=LINE('',#226408,#28436);
#23210=LINE('',#226410,#28437);
#23211=LINE('',#226414,#28438);
#23212=LINE('',#226418,#28439);
#23213=LINE('',#226419,#28440);
#23214=LINE('',#226425,#28441);
#23215=LINE('',#226427,#28442);
#23216=LINE('',#226429,#28443);
#23217=LINE('',#226433,#28444);
#23218=LINE('',#226435,#28445);
#23219=LINE('',#226439,#28446);
#23220=LINE('',#226443,#28447);
#23221=LINE('',#226444,#28448);
#23222=LINE('',#226448,#28449);
#23223=LINE('',#226452,#28450);
#23224=LINE('',#226459,#28451);
#23225=LINE('',#226461,#28452);
#23226=LINE('',#226463,#28453);
#23227=LINE('',#226467,#28454);
#23228=LINE('',#226469,#28455);
#23229=LINE('',#226473,#28456);
#23230=LINE('',#226477,#28457);
#23231=LINE('',#226478,#28458);
#23232=LINE('',#226484,#28459);
#23233=LINE('',#226486,#28460);
#23234=LINE('',#226488,#28461);
#23235=LINE('',#226492,#28462);
#23236=LINE('',#226494,#28463);
#23237=LINE('',#226498,#28464);
#23238=LINE('',#226502,#28465);
#23239=LINE('',#226503,#28466);
#23240=LINE('',#226507,#28467);
#23241=LINE('',#226511,#28468);
#23242=LINE('',#226518,#28469);
#23243=LINE('',#226520,#28470);
#23244=LINE('',#226522,#28471);
#23245=LINE('',#226526,#28472);
#23246=LINE('',#226528,#28473);
#23247=LINE('',#226532,#28474);
#23248=LINE('',#226536,#28475);
#23249=LINE('',#226537,#28476);
#23250=LINE('',#226543,#28477);
#23251=LINE('',#226545,#28478);
#23252=LINE('',#226547,#28479);
#23253=LINE('',#226551,#28480);
#23254=LINE('',#226553,#28481);
#23255=LINE('',#226557,#28482);
#23256=LINE('',#226561,#28483);
#23257=LINE('',#226562,#28484);
#23258=LINE('',#226566,#28485);
#23259=LINE('',#226570,#28486);
#23260=LINE('',#226577,#28487);
#23261=LINE('',#226579,#28488);
#23262=LINE('',#226581,#28489);
#23263=LINE('',#226585,#28490);
#23264=LINE('',#226587,#28491);
#23265=LINE('',#226591,#28492);
#23266=LINE('',#226595,#28493);
#23267=LINE('',#226596,#28494);
#23268=LINE('',#226602,#28495);
#23269=LINE('',#226604,#28496);
#23270=LINE('',#226606,#28497);
#23271=LINE('',#226610,#28498);
#23272=LINE('',#226612,#28499);
#23273=LINE('',#226616,#28500);
#23274=LINE('',#226620,#28501);
#23275=LINE('',#226621,#28502);
#23276=LINE('',#226625,#28503);
#23277=LINE('',#226629,#28504);
#23278=LINE('',#226636,#28505);
#23279=LINE('',#226638,#28506);
#23280=LINE('',#226640,#28507);
#23281=LINE('',#226644,#28508);
#23282=LINE('',#226646,#28509);
#23283=LINE('',#226650,#28510);
#23284=LINE('',#226654,#28511);
#23285=LINE('',#226655,#28512);
#23286=LINE('',#226661,#28513);
#23287=LINE('',#226663,#28514);
#23288=LINE('',#226665,#28515);
#23289=LINE('',#226669,#28516);
#23290=LINE('',#226671,#28517);
#23291=LINE('',#226675,#28518);
#23292=LINE('',#226679,#28519);
#23293=LINE('',#226680,#28520);
#23294=LINE('',#226684,#28521);
#23295=LINE('',#226688,#28522);
#23296=LINE('',#226695,#28523);
#23297=LINE('',#226697,#28524);
#23298=LINE('',#226699,#28525);
#23299=LINE('',#226703,#28526);
#23300=LINE('',#226705,#28527);
#23301=LINE('',#226709,#28528);
#23302=LINE('',#226713,#28529);
#23303=LINE('',#226714,#28530);
#23304=LINE('',#226720,#28531);
#23305=LINE('',#226722,#28532);
#23306=LINE('',#226724,#28533);
#23307=LINE('',#226728,#28534);
#23308=LINE('',#226730,#28535);
#23309=LINE('',#226734,#28536);
#23310=LINE('',#226738,#28537);
#23311=LINE('',#226739,#28538);
#23312=LINE('',#226743,#28539);
#23313=LINE('',#226747,#28540);
#23314=LINE('',#226754,#28541);
#23315=LINE('',#226756,#28542);
#23316=LINE('',#226758,#28543);
#23317=LINE('',#226762,#28544);
#23318=LINE('',#226764,#28545);
#23319=LINE('',#226768,#28546);
#23320=LINE('',#226772,#28547);
#23321=LINE('',#226773,#28548);
#23322=LINE('',#226779,#28549);
#23323=LINE('',#226781,#28550);
#23324=LINE('',#226783,#28551);
#23325=LINE('',#226787,#28552);
#23326=LINE('',#226789,#28553);
#23327=LINE('',#226793,#28554);
#23328=LINE('',#226797,#28555);
#23329=LINE('',#226798,#28556);
#23330=LINE('',#226802,#28557);
#23331=LINE('',#226806,#28558);
#23332=LINE('',#226813,#28559);
#23333=LINE('',#226815,#28560);
#23334=LINE('',#226817,#28561);
#23335=LINE('',#226821,#28562);
#23336=LINE('',#226823,#28563);
#23337=LINE('',#226827,#28564);
#23338=LINE('',#226831,#28565);
#23339=LINE('',#226832,#28566);
#23340=LINE('',#226838,#28567);
#23341=LINE('',#226840,#28568);
#23342=LINE('',#226842,#28569);
#23343=LINE('',#226846,#28570);
#23344=LINE('',#226848,#28571);
#23345=LINE('',#226852,#28572);
#23346=LINE('',#226856,#28573);
#23347=LINE('',#226857,#28574);
#23348=LINE('',#226861,#28575);
#23349=LINE('',#226865,#28576);
#23350=LINE('',#226872,#28577);
#23351=LINE('',#226874,#28578);
#23352=LINE('',#226876,#28579);
#23353=LINE('',#226880,#28580);
#23354=LINE('',#226882,#28581);
#23355=LINE('',#226886,#28582);
#23356=LINE('',#226890,#28583);
#23357=LINE('',#226891,#28584);
#23358=LINE('',#226897,#28585);
#23359=LINE('',#226899,#28586);
#23360=LINE('',#226901,#28587);
#23361=LINE('',#226905,#28588);
#23362=LINE('',#226907,#28589);
#23363=LINE('',#226911,#28590);
#23364=LINE('',#226915,#28591);
#23365=LINE('',#226916,#28592);
#23366=LINE('',#226920,#28593);
#23367=LINE('',#226924,#28594);
#23368=LINE('',#226931,#28595);
#23369=LINE('',#226933,#28596);
#23370=LINE('',#226935,#28597);
#23371=LINE('',#226939,#28598);
#23372=LINE('',#226941,#28599);
#23373=LINE('',#226945,#28600);
#23374=LINE('',#226949,#28601);
#23375=LINE('',#226950,#28602);
#23376=LINE('',#226956,#28603);
#23377=LINE('',#226958,#28604);
#23378=LINE('',#226960,#28605);
#23379=LINE('',#226964,#28606);
#23380=LINE('',#226966,#28607);
#23381=LINE('',#226970,#28608);
#23382=LINE('',#226974,#28609);
#23383=LINE('',#226975,#28610);
#23384=LINE('',#226979,#28611);
#23385=LINE('',#226983,#28612);
#23386=LINE('',#226990,#28613);
#23387=LINE('',#226992,#28614);
#23388=LINE('',#226994,#28615);
#23389=LINE('',#226998,#28616);
#23390=LINE('',#227000,#28617);
#23391=LINE('',#227004,#28618);
#23392=LINE('',#227008,#28619);
#23393=LINE('',#227009,#28620);
#23394=LINE('',#227015,#28621);
#23395=LINE('',#227017,#28622);
#23396=LINE('',#227019,#28623);
#23397=LINE('',#227023,#28624);
#23398=LINE('',#227025,#28625);
#23399=LINE('',#227029,#28626);
#23400=LINE('',#227033,#28627);
#23401=LINE('',#227034,#28628);
#23402=LINE('',#227038,#28629);
#23403=LINE('',#227042,#28630);
#23404=LINE('',#227049,#28631);
#23405=LINE('',#227051,#28632);
#23406=LINE('',#227053,#28633);
#23407=LINE('',#227057,#28634);
#23408=LINE('',#227059,#28635);
#23409=LINE('',#227063,#28636);
#23410=LINE('',#227067,#28637);
#23411=LINE('',#227068,#28638);
#23412=LINE('',#227074,#28639);
#23413=LINE('',#227076,#28640);
#23414=LINE('',#227078,#28641);
#23415=LINE('',#227082,#28642);
#23416=LINE('',#227084,#28643);
#23417=LINE('',#227088,#28644);
#23418=LINE('',#227092,#28645);
#23419=LINE('',#227093,#28646);
#23420=LINE('',#227095,#28647);
#23421=LINE('',#227096,#28648);
#23422=LINE('',#227102,#28649);
#23423=LINE('',#227104,#28650);
#23424=LINE('',#227106,#28651);
#23425=LINE('',#227110,#28652);
#23426=LINE('',#227112,#28653);
#23427=LINE('',#227116,#28654);
#23428=LINE('',#227120,#28655);
#23429=LINE('',#227121,#28656);
#23430=LINE('',#227127,#28657);
#23431=LINE('',#227129,#28658);
#23432=LINE('',#227131,#28659);
#23433=LINE('',#227135,#28660);
#23434=LINE('',#227137,#28661);
#23435=LINE('',#227141,#28662);
#23436=LINE('',#227145,#28663);
#23437=LINE('',#227146,#28664);
#23438=LINE('',#227150,#28665);
#23439=LINE('',#227154,#28666);
#23440=LINE('',#227161,#28667);
#23441=LINE('',#227163,#28668);
#23442=LINE('',#227165,#28669);
#23443=LINE('',#227169,#28670);
#23444=LINE('',#227171,#28671);
#23445=LINE('',#227175,#28672);
#23446=LINE('',#227179,#28673);
#23447=LINE('',#227180,#28674);
#23448=LINE('',#227186,#28675);
#23449=LINE('',#227188,#28676);
#23450=LINE('',#227190,#28677);
#23451=LINE('',#227194,#28678);
#23452=LINE('',#227196,#28679);
#23453=LINE('',#227200,#28680);
#23454=LINE('',#227204,#28681);
#23455=LINE('',#227205,#28682);
#23456=LINE('',#227209,#28683);
#23457=LINE('',#227213,#28684);
#23458=LINE('',#227220,#28685);
#23459=LINE('',#227222,#28686);
#23460=LINE('',#227224,#28687);
#23461=LINE('',#227228,#28688);
#23462=LINE('',#227230,#28689);
#23463=LINE('',#227234,#28690);
#23464=LINE('',#227238,#28691);
#23465=LINE('',#227239,#28692);
#23466=LINE('',#227245,#28693);
#23467=LINE('',#227247,#28694);
#23468=LINE('',#227249,#28695);
#23469=LINE('',#227253,#28696);
#23470=LINE('',#227255,#28697);
#23471=LINE('',#227259,#28698);
#23472=LINE('',#227263,#28699);
#23473=LINE('',#227264,#28700);
#23474=LINE('',#227268,#28701);
#23475=LINE('',#227272,#28702);
#23476=LINE('',#227279,#28703);
#23477=LINE('',#227281,#28704);
#23478=LINE('',#227283,#28705);
#23479=LINE('',#227287,#28706);
#23480=LINE('',#227289,#28707);
#23481=LINE('',#227293,#28708);
#23482=LINE('',#227297,#28709);
#23483=LINE('',#227298,#28710);
#23484=LINE('',#227304,#28711);
#23485=LINE('',#227306,#28712);
#23486=LINE('',#227308,#28713);
#23487=LINE('',#227312,#28714);
#23488=LINE('',#227314,#28715);
#23489=LINE('',#227318,#28716);
#23490=LINE('',#227322,#28717);
#23491=LINE('',#227323,#28718);
#23492=LINE('',#227327,#28719);
#23493=LINE('',#227331,#28720);
#23494=LINE('',#227338,#28721);
#23495=LINE('',#227340,#28722);
#23496=LINE('',#227342,#28723);
#23497=LINE('',#227346,#28724);
#23498=LINE('',#227348,#28725);
#23499=LINE('',#227352,#28726);
#23500=LINE('',#227356,#28727);
#23501=LINE('',#227357,#28728);
#23502=LINE('',#227363,#28729);
#23503=LINE('',#227365,#28730);
#23504=LINE('',#227367,#28731);
#23505=LINE('',#227371,#28732);
#23506=LINE('',#227373,#28733);
#23507=LINE('',#227377,#28734);
#23508=LINE('',#227381,#28735);
#23509=LINE('',#227382,#28736);
#23510=LINE('',#227386,#28737);
#23511=LINE('',#227390,#28738);
#23512=LINE('',#227397,#28739);
#23513=LINE('',#227399,#28740);
#23514=LINE('',#227401,#28741);
#23515=LINE('',#227405,#28742);
#23516=LINE('',#227407,#28743);
#23517=LINE('',#227411,#28744);
#23518=LINE('',#227415,#28745);
#23519=LINE('',#227416,#28746);
#23520=LINE('',#227422,#28747);
#23521=LINE('',#227424,#28748);
#23522=LINE('',#227426,#28749);
#23523=LINE('',#227430,#28750);
#23524=LINE('',#227432,#28751);
#23525=LINE('',#227436,#28752);
#23526=LINE('',#227440,#28753);
#23527=LINE('',#227441,#28754);
#23528=LINE('',#227445,#28755);
#23529=LINE('',#227449,#28756);
#23530=LINE('',#227456,#28757);
#23531=LINE('',#227458,#28758);
#23532=LINE('',#227460,#28759);
#23533=LINE('',#227464,#28760);
#23534=LINE('',#227466,#28761);
#23535=LINE('',#227470,#28762);
#23536=LINE('',#227474,#28763);
#23537=LINE('',#227475,#28764);
#23538=LINE('',#227481,#28765);
#23539=LINE('',#227483,#28766);
#23540=LINE('',#227485,#28767);
#23541=LINE('',#227489,#28768);
#23542=LINE('',#227491,#28769);
#23543=LINE('',#227495,#28770);
#23544=LINE('',#227499,#28771);
#23545=LINE('',#227500,#28772);
#23546=LINE('',#227504,#28773);
#23547=LINE('',#227508,#28774);
#23548=LINE('',#227515,#28775);
#23549=LINE('',#227517,#28776);
#23550=LINE('',#227519,#28777);
#23551=LINE('',#227523,#28778);
#23552=LINE('',#227525,#28779);
#23553=LINE('',#227529,#28780);
#23554=LINE('',#227533,#28781);
#23555=LINE('',#227534,#28782);
#23556=LINE('',#227540,#28783);
#23557=LINE('',#227542,#28784);
#23558=LINE('',#227544,#28785);
#23559=LINE('',#227548,#28786);
#23560=LINE('',#227550,#28787);
#23561=LINE('',#227554,#28788);
#23562=LINE('',#227558,#28789);
#23563=LINE('',#227559,#28790);
#23564=LINE('',#227563,#28791);
#23565=LINE('',#227567,#28792);
#23566=LINE('',#227574,#28793);
#23567=LINE('',#227576,#28794);
#23568=LINE('',#227578,#28795);
#23569=LINE('',#227582,#28796);
#23570=LINE('',#227584,#28797);
#23571=LINE('',#227588,#28798);
#23572=LINE('',#227592,#28799);
#23573=LINE('',#227593,#28800);
#23574=LINE('',#227599,#28801);
#23575=LINE('',#227601,#28802);
#23576=LINE('',#227603,#28803);
#23577=LINE('',#227607,#28804);
#23578=LINE('',#227609,#28805);
#23579=LINE('',#227613,#28806);
#23580=LINE('',#227617,#28807);
#23581=LINE('',#227618,#28808);
#23582=LINE('',#227622,#28809);
#23583=LINE('',#227626,#28810);
#23584=LINE('',#227633,#28811);
#23585=LINE('',#227635,#28812);
#23586=LINE('',#227637,#28813);
#23587=LINE('',#227641,#28814);
#23588=LINE('',#227643,#28815);
#23589=LINE('',#227647,#28816);
#23590=LINE('',#227651,#28817);
#23591=LINE('',#227652,#28818);
#23592=LINE('',#227658,#28819);
#23593=LINE('',#227660,#28820);
#23594=LINE('',#227662,#28821);
#23595=LINE('',#227666,#28822);
#23596=LINE('',#227668,#28823);
#23597=LINE('',#227672,#28824);
#23598=LINE('',#227676,#28825);
#23599=LINE('',#227677,#28826);
#23600=LINE('',#227681,#28827);
#23601=LINE('',#227685,#28828);
#23602=LINE('',#227692,#28829);
#23603=LINE('',#227694,#28830);
#23604=LINE('',#227696,#28831);
#23605=LINE('',#227700,#28832);
#23606=LINE('',#227702,#28833);
#23607=LINE('',#227706,#28834);
#23608=LINE('',#227710,#28835);
#23609=LINE('',#227711,#28836);
#23610=LINE('',#227717,#28837);
#23611=LINE('',#227719,#28838);
#23612=LINE('',#227721,#28839);
#23613=LINE('',#227725,#28840);
#23614=LINE('',#227727,#28841);
#23615=LINE('',#227731,#28842);
#23616=LINE('',#227735,#28843);
#23617=LINE('',#227736,#28844);
#23618=LINE('',#227740,#28845);
#23619=LINE('',#227744,#28846);
#23620=LINE('',#227751,#28847);
#23621=LINE('',#227753,#28848);
#23622=LINE('',#227755,#28849);
#23623=LINE('',#227759,#28850);
#23624=LINE('',#227761,#28851);
#23625=LINE('',#227765,#28852);
#23626=LINE('',#227769,#28853);
#23627=LINE('',#227770,#28854);
#23628=LINE('',#227776,#28855);
#23629=LINE('',#227778,#28856);
#23630=LINE('',#227780,#28857);
#23631=LINE('',#227784,#28858);
#23632=LINE('',#227786,#28859);
#23633=LINE('',#227790,#28860);
#23634=LINE('',#227794,#28861);
#23635=LINE('',#227795,#28862);
#23636=LINE('',#227799,#28863);
#23637=LINE('',#227803,#28864);
#23638=LINE('',#227810,#28865);
#23639=LINE('',#227812,#28866);
#23640=LINE('',#227814,#28867);
#23641=LINE('',#227818,#28868);
#23642=LINE('',#227820,#28869);
#23643=LINE('',#227824,#28870);
#23644=LINE('',#227828,#28871);
#23645=LINE('',#227829,#28872);
#23646=LINE('',#227835,#28873);
#23647=LINE('',#227837,#28874);
#23648=LINE('',#227839,#28875);
#23649=LINE('',#227843,#28876);
#23650=LINE('',#227845,#28877);
#23651=LINE('',#227849,#28878);
#23652=LINE('',#227853,#28879);
#23653=LINE('',#227854,#28880);
#23654=LINE('',#227858,#28881);
#23655=LINE('',#227862,#28882);
#23656=LINE('',#227869,#28883);
#23657=LINE('',#227871,#28884);
#23658=LINE('',#227873,#28885);
#23659=LINE('',#227877,#28886);
#23660=LINE('',#227879,#28887);
#23661=LINE('',#227883,#28888);
#23662=LINE('',#227887,#28889);
#23663=LINE('',#227888,#28890);
#23664=LINE('',#227894,#28891);
#23665=LINE('',#227896,#28892);
#23666=LINE('',#227898,#28893);
#23667=LINE('',#227902,#28894);
#23668=LINE('',#227904,#28895);
#23669=LINE('',#227908,#28896);
#23670=LINE('',#227912,#28897);
#23671=LINE('',#227913,#28898);
#23672=LINE('',#227917,#28899);
#23673=LINE('',#227921,#28900);
#23674=LINE('',#227928,#28901);
#23675=LINE('',#227930,#28902);
#23676=LINE('',#227932,#28903);
#23677=LINE('',#227936,#28904);
#23678=LINE('',#227938,#28905);
#23679=LINE('',#227942,#28906);
#23680=LINE('',#227946,#28907);
#23681=LINE('',#227947,#28908);
#23682=LINE('',#227953,#28909);
#23683=LINE('',#227955,#28910);
#23684=LINE('',#227957,#28911);
#23685=LINE('',#227961,#28912);
#23686=LINE('',#227963,#28913);
#23687=LINE('',#227967,#28914);
#23688=LINE('',#227971,#28915);
#23689=LINE('',#227972,#28916);
#23690=LINE('',#227974,#28917);
#23691=LINE('',#227975,#28918);
#23692=LINE('',#227981,#28919);
#23693=LINE('',#227983,#28920);
#23694=LINE('',#227985,#28921);
#23695=LINE('',#227989,#28922);
#23696=LINE('',#227991,#28923);
#23697=LINE('',#227995,#28924);
#23698=LINE('',#227999,#28925);
#23699=LINE('',#228000,#28926);
#23700=LINE('',#228006,#28927);
#23701=LINE('',#228008,#28928);
#23702=LINE('',#228010,#28929);
#23703=LINE('',#228014,#28930);
#23704=LINE('',#228016,#28931);
#23705=LINE('',#228020,#28932);
#23706=LINE('',#228024,#28933);
#23707=LINE('',#228025,#28934);
#23708=LINE('',#228029,#28935);
#23709=LINE('',#228033,#28936);
#23710=LINE('',#228040,#28937);
#23711=LINE('',#228042,#28938);
#23712=LINE('',#228044,#28939);
#23713=LINE('',#228048,#28940);
#23714=LINE('',#228050,#28941);
#23715=LINE('',#228054,#28942);
#23716=LINE('',#228058,#28943);
#23717=LINE('',#228059,#28944);
#23718=LINE('',#228065,#28945);
#23719=LINE('',#228067,#28946);
#23720=LINE('',#228069,#28947);
#23721=LINE('',#228073,#28948);
#23722=LINE('',#228075,#28949);
#23723=LINE('',#228079,#28950);
#23724=LINE('',#228083,#28951);
#23725=LINE('',#228084,#28952);
#23726=LINE('',#228088,#28953);
#23727=LINE('',#228092,#28954);
#23728=LINE('',#228099,#28955);
#23729=LINE('',#228101,#28956);
#23730=LINE('',#228103,#28957);
#23731=LINE('',#228107,#28958);
#23732=LINE('',#228109,#28959);
#23733=LINE('',#228113,#28960);
#23734=LINE('',#228117,#28961);
#23735=LINE('',#228118,#28962);
#23736=LINE('',#228124,#28963);
#23737=LINE('',#228126,#28964);
#23738=LINE('',#228128,#28965);
#23739=LINE('',#228132,#28966);
#23740=LINE('',#228134,#28967);
#23741=LINE('',#228138,#28968);
#23742=LINE('',#228142,#28969);
#23743=LINE('',#228143,#28970);
#23744=LINE('',#228147,#28971);
#23745=LINE('',#228151,#28972);
#23746=LINE('',#228158,#28973);
#23747=LINE('',#228160,#28974);
#23748=LINE('',#228162,#28975);
#23749=LINE('',#228166,#28976);
#23750=LINE('',#228168,#28977);
#23751=LINE('',#228172,#28978);
#23752=LINE('',#228176,#28979);
#23753=LINE('',#228177,#28980);
#23754=LINE('',#228183,#28981);
#23755=LINE('',#228185,#28982);
#23756=LINE('',#228187,#28983);
#23757=LINE('',#228191,#28984);
#23758=LINE('',#228193,#28985);
#23759=LINE('',#228197,#28986);
#23760=LINE('',#228201,#28987);
#23761=LINE('',#228202,#28988);
#23762=LINE('',#228206,#28989);
#23763=LINE('',#228210,#28990);
#23764=LINE('',#228217,#28991);
#23765=LINE('',#228219,#28992);
#23766=LINE('',#228221,#28993);
#23767=LINE('',#228225,#28994);
#23768=LINE('',#228227,#28995);
#23769=LINE('',#228231,#28996);
#23770=LINE('',#228235,#28997);
#23771=LINE('',#228236,#28998);
#23772=LINE('',#228242,#28999);
#23773=LINE('',#228244,#29000);
#23774=LINE('',#228246,#29001);
#23775=LINE('',#228250,#29002);
#23776=LINE('',#228252,#29003);
#23777=LINE('',#228256,#29004);
#23778=LINE('',#228260,#29005);
#23779=LINE('',#228261,#29006);
#23780=LINE('',#228265,#29007);
#23781=LINE('',#228269,#29008);
#23782=LINE('',#228276,#29009);
#23783=LINE('',#228278,#29010);
#23784=LINE('',#228280,#29011);
#23785=LINE('',#228284,#29012);
#23786=LINE('',#228286,#29013);
#23787=LINE('',#228290,#29014);
#23788=LINE('',#228294,#29015);
#23789=LINE('',#228295,#29016);
#23790=LINE('',#228301,#29017);
#23791=LINE('',#228303,#29018);
#23792=LINE('',#228305,#29019);
#23793=LINE('',#228309,#29020);
#23794=LINE('',#228311,#29021);
#23795=LINE('',#228315,#29022);
#23796=LINE('',#228319,#29023);
#23797=LINE('',#228320,#29024);
#23798=LINE('',#228324,#29025);
#23799=LINE('',#228328,#29026);
#23800=LINE('',#228335,#29027);
#23801=LINE('',#228337,#29028);
#23802=LINE('',#228339,#29029);
#23803=LINE('',#228343,#29030);
#23804=LINE('',#228345,#29031);
#23805=LINE('',#228349,#29032);
#23806=LINE('',#228353,#29033);
#23807=LINE('',#228354,#29034);
#23808=LINE('',#228360,#29035);
#23809=LINE('',#228362,#29036);
#23810=LINE('',#228364,#29037);
#23811=LINE('',#228368,#29038);
#23812=LINE('',#228370,#29039);
#23813=LINE('',#228374,#29040);
#23814=LINE('',#228378,#29041);
#23815=LINE('',#228379,#29042);
#23816=LINE('',#228383,#29043);
#23817=LINE('',#228387,#29044);
#23818=LINE('',#228394,#29045);
#23819=LINE('',#228396,#29046);
#23820=LINE('',#228398,#29047);
#23821=LINE('',#228402,#29048);
#23822=LINE('',#228404,#29049);
#23823=LINE('',#228408,#29050);
#23824=LINE('',#228412,#29051);
#23825=LINE('',#228413,#29052);
#23826=LINE('',#228419,#29053);
#23827=LINE('',#228421,#29054);
#23828=LINE('',#228423,#29055);
#23829=LINE('',#228427,#29056);
#23830=LINE('',#228429,#29057);
#23831=LINE('',#228433,#29058);
#23832=LINE('',#228437,#29059);
#23833=LINE('',#228438,#29060);
#23834=LINE('',#228442,#29061);
#23835=LINE('',#228446,#29062);
#23836=LINE('',#228453,#29063);
#23837=LINE('',#228455,#29064);
#23838=LINE('',#228457,#29065);
#23839=LINE('',#228461,#29066);
#23840=LINE('',#228463,#29067);
#23841=LINE('',#228467,#29068);
#23842=LINE('',#228471,#29069);
#23843=LINE('',#228472,#29070);
#23844=LINE('',#228478,#29071);
#23845=LINE('',#228480,#29072);
#23846=LINE('',#228482,#29073);
#23847=LINE('',#228486,#29074);
#23848=LINE('',#228488,#29075);
#23849=LINE('',#228492,#29076);
#23850=LINE('',#228496,#29077);
#23851=LINE('',#228497,#29078);
#23852=LINE('',#228501,#29079);
#23853=LINE('',#228505,#29080);
#23854=LINE('',#228512,#29081);
#23855=LINE('',#228514,#29082);
#23856=LINE('',#228516,#29083);
#23857=LINE('',#228520,#29084);
#23858=LINE('',#228522,#29085);
#23859=LINE('',#228526,#29086);
#23860=LINE('',#228530,#29087);
#23861=LINE('',#228531,#29088);
#23862=LINE('',#228537,#29089);
#23863=LINE('',#228539,#29090);
#23864=LINE('',#228541,#29091);
#23865=LINE('',#228545,#29092);
#23866=LINE('',#228547,#29093);
#23867=LINE('',#228551,#29094);
#23868=LINE('',#228555,#29095);
#23869=LINE('',#228556,#29096);
#23870=LINE('',#228560,#29097);
#23871=LINE('',#228564,#29098);
#23872=LINE('',#228571,#29099);
#23873=LINE('',#228573,#29100);
#23874=LINE('',#228575,#29101);
#23875=LINE('',#228579,#29102);
#23876=LINE('',#228581,#29103);
#23877=LINE('',#228585,#29104);
#23878=LINE('',#228589,#29105);
#23879=LINE('',#228590,#29106);
#23880=LINE('',#228596,#29107);
#23881=LINE('',#228598,#29108);
#23882=LINE('',#228600,#29109);
#23883=LINE('',#228604,#29110);
#23884=LINE('',#228606,#29111);
#23885=LINE('',#228610,#29112);
#23886=LINE('',#228614,#29113);
#23887=LINE('',#228615,#29114);
#23888=LINE('',#228619,#29115);
#23889=LINE('',#228623,#29116);
#23890=LINE('',#228630,#29117);
#23891=LINE('',#228632,#29118);
#23892=LINE('',#228634,#29119);
#23893=LINE('',#228638,#29120);
#23894=LINE('',#228640,#29121);
#23895=LINE('',#228644,#29122);
#23896=LINE('',#228648,#29123);
#23897=LINE('',#228649,#29124);
#23898=LINE('',#228655,#29125);
#23899=LINE('',#228657,#29126);
#23900=LINE('',#228659,#29127);
#23901=LINE('',#228663,#29128);
#23902=LINE('',#228665,#29129);
#23903=LINE('',#228669,#29130);
#23904=LINE('',#228673,#29131);
#23905=LINE('',#228674,#29132);
#23906=LINE('',#228678,#29133);
#23907=LINE('',#228682,#29134);
#23908=LINE('',#228689,#29135);
#23909=LINE('',#228691,#29136);
#23910=LINE('',#228693,#29137);
#23911=LINE('',#228697,#29138);
#23912=LINE('',#228699,#29139);
#23913=LINE('',#228703,#29140);
#23914=LINE('',#228707,#29141);
#23915=LINE('',#228708,#29142);
#23916=LINE('',#228714,#29143);
#23917=LINE('',#228716,#29144);
#23918=LINE('',#228718,#29145);
#23919=LINE('',#228722,#29146);
#23920=LINE('',#228724,#29147);
#23921=LINE('',#228728,#29148);
#23922=LINE('',#228732,#29149);
#23923=LINE('',#228733,#29150);
#23924=LINE('',#228737,#29151);
#23925=LINE('',#228741,#29152);
#23926=LINE('',#228748,#29153);
#23927=LINE('',#228750,#29154);
#23928=LINE('',#228752,#29155);
#23929=LINE('',#228756,#29156);
#23930=LINE('',#228758,#29157);
#23931=LINE('',#228762,#29158);
#23932=LINE('',#228766,#29159);
#23933=LINE('',#228767,#29160);
#23934=LINE('',#228773,#29161);
#23935=LINE('',#228775,#29162);
#23936=LINE('',#228777,#29163);
#23937=LINE('',#228781,#29164);
#23938=LINE('',#228783,#29165);
#23939=LINE('',#228787,#29166);
#23940=LINE('',#228791,#29167);
#23941=LINE('',#228792,#29168);
#23942=LINE('',#228796,#29169);
#23943=LINE('',#228800,#29170);
#23944=LINE('',#228807,#29171);
#23945=LINE('',#228809,#29172);
#23946=LINE('',#228811,#29173);
#23947=LINE('',#228815,#29174);
#23948=LINE('',#228817,#29175);
#23949=LINE('',#228821,#29176);
#23950=LINE('',#228825,#29177);
#23951=LINE('',#228826,#29178);
#23952=LINE('',#228832,#29179);
#23953=LINE('',#228834,#29180);
#23954=LINE('',#228836,#29181);
#23955=LINE('',#228840,#29182);
#23956=LINE('',#228842,#29183);
#23957=LINE('',#228846,#29184);
#23958=LINE('',#228850,#29185);
#23959=LINE('',#228851,#29186);
#23960=LINE('',#253407,#29187);
#23961=LINE('',#253409,#29188);
#23962=LINE('',#253414,#29189);
#23963=LINE('',#253434,#29190);
#23964=LINE('',#253437,#29191);
#23965=LINE('',#253547,#29192);
#23966=LINE('',#253578,#29193);
#23967=LINE('',#253581,#29194);
#23968=LINE('',#253630,#29195);
#23969=LINE('',#253648,#29196);
#23970=LINE('',#253654,#29197);
#23971=LINE('',#253660,#29198);
#23972=LINE('',#253666,#29199);
#23973=LINE('',#253672,#29200);
#23974=LINE('',#253676,#29201);
#23975=LINE('',#253679,#29202);
#23976=LINE('',#254180,#29203);
#23977=LINE('',#254191,#29204);
#23978=LINE('',#254195,#29205);
#23979=LINE('',#254251,#29206);
#23980=LINE('',#254257,#29207);
#23981=LINE('',#254320,#29208);
#23982=LINE('',#254324,#29209);
#23983=LINE('',#254380,#29210);
#23984=LINE('',#254384,#29211);
#23985=LINE('',#254385,#29212);
#23986=LINE('',#254386,#29213);
#23987=LINE('',#254388,#29214);
#23988=LINE('',#254389,#29215);
#23989=LINE('',#254393,#29216);
#23990=LINE('',#254395,#29217);
#23991=LINE('',#254397,#29218);
#23992=LINE('',#254398,#29219);
#23993=LINE('',#254401,#29220);
#23994=LINE('',#254403,#29221);
#23995=LINE('',#254521,#29222);
#23996=LINE('',#254523,#29223);
#23997=LINE('',#254587,#29224);
#23998=LINE('',#254657,#29225);
#23999=LINE('',#254658,#29226);
#24000=LINE('',#254659,#29227);
#24001=LINE('',#254663,#29228);
#24002=LINE('',#254667,#29229);
#24003=LINE('',#254671,#29230);
#24004=LINE('',#254673,#29231);
#24005=LINE('',#254674,#29232);
#24006=LINE('',#254679,#29233);
#24007=LINE('',#254683,#29234);
#24008=LINE('',#254685,#29235);
#24009=LINE('',#254686,#29236);
#24010=LINE('',#254691,#29237);
#24011=LINE('',#254695,#29238);
#24012=LINE('',#254697,#29239);
#24013=LINE('',#254698,#29240);
#24014=LINE('',#254703,#29241);
#24015=LINE('',#254706,#29242);
#24016=LINE('',#254707,#29243);
#24017=LINE('',#254757,#29244);
#24018=LINE('',#254761,#29245);
#24019=LINE('',#254816,#29246);
#24020=LINE('',#254818,#29247);
#24021=LINE('',#254846,#29248);
#24022=LINE('',#254851,#29249);
#24023=LINE('',#254853,#29250);
#24024=LINE('',#254862,#29251);
#24025=LINE('',#254998,#29252);
#24026=LINE('',#255001,#29253);
#24027=LINE('',#255004,#29254);
#24028=LINE('',#255025,#29255);
#24029=LINE('',#255044,#29256);
#24030=LINE('',#255046,#29257);
#24031=LINE('',#255054,#29258);
#24032=LINE('',#255055,#29259);
#24033=LINE('',#255059,#29260);
#24034=LINE('',#255063,#29261);
#24035=LINE('',#255070,#29262);
#24036=LINE('',#255074,#29263);
#24037=LINE('',#255079,#29264);
#24038=LINE('',#255083,#29265);
#24039=LINE('',#255087,#29266);
#24040=LINE('',#255090,#29267);
#24041=LINE('',#255093,#29268);
#24042=LINE('',#255096,#29269);
#24043=LINE('',#255099,#29270);
#24044=LINE('',#255161,#29271);
#24045=LINE('',#255164,#29272);
#24046=LINE('',#255223,#29273);
#24047=LINE('',#255286,#29274);
#24048=LINE('',#255287,#29275);
#24049=LINE('',#255293,#29276);
#24050=LINE('',#255296,#29277);
#24051=LINE('',#255298,#29278);
#24052=LINE('',#255301,#29279);
#24053=LINE('',#255359,#29280);
#24054=LINE('',#255363,#29281);
#24055=LINE('',#255425,#29282);
#24056=LINE('',#255426,#29283);
#24057=LINE('',#255432,#29284);
#24058=LINE('',#255436,#29285);
#24059=LINE('',#255443,#29286);
#24060=LINE('',#255446,#29287);
#24061=LINE('',#255506,#29288);
#24062=LINE('',#255507,#29289);
#24063=LINE('',#255510,#29290);
#24064=LINE('',#255572,#29291);
#24065=LINE('',#255573,#29292);
#24066=LINE('',#255579,#29293);
#24067=LINE('',#255582,#29294);
#24068=LINE('',#255583,#29295);
#24069=LINE('',#255586,#29296);
#24070=LINE('',#255589,#29297);
#24071=LINE('',#255590,#29298);
#24072=LINE('',#261328,#29299);
#24073=LINE('',#261411,#29300);
#24074=LINE('',#261529,#29301);
#24075=LINE('',#261571,#29302);
#24076=LINE('',#261574,#29303);
#24077=LINE('',#261616,#29304);
#24078=LINE('',#261619,#29305);
#24079=LINE('',#261621,#29306);
#24080=LINE('',#261625,#29307);
#24081=LINE('',#261628,#29308);
#24082=LINE('',#261634,#29309);
#24083=LINE('',#261644,#29310);
#24084=LINE('',#261681,#29311);
#24085=LINE('',#261719,#29312);
#24086=LINE('',#261757,#29313);
#24087=LINE('',#261795,#29314);
#24088=LINE('',#261833,#29315);
#24089=LINE('',#261871,#29316);
#24090=LINE('',#261887,#29317);
#24091=LINE('',#261941,#29318);
#24092=LINE('',#262017,#29319);
#24093=LINE('',#262093,#29320);
#24094=LINE('',#262169,#29321);
#24095=LINE('',#262245,#29322);
#24096=LINE('',#262323,#29323);
#24097=LINE('',#262393,#29324);
#24098=LINE('',#262403,#29325);
#24099=LINE('',#262467,#29326);
#24100=LINE('',#262469,#29327);
#24101=LINE('',#262471,#29328);
#24102=LINE('',#262473,#29329);
#24103=LINE('',#262475,#29330);
#24104=LINE('',#262476,#29331);
#24105=LINE('',#262478,#29332);
#24106=LINE('',#262479,#29333);
#24107=LINE('',#262481,#29334);
#24108=LINE('',#262483,#29335);
#24109=LINE('',#262485,#29336);
#24110=LINE('',#262487,#29337);
#24111=LINE('',#263171,#29338);
#24112=LINE('',#263208,#29339);
#24113=LINE('',#263246,#29340);
#24114=LINE('',#263284,#29341);
#24115=LINE('',#263322,#29342);
#24116=LINE('',#263360,#29343);
#24117=LINE('',#263398,#29344);
#24118=LINE('',#263414,#29345);
#24119=LINE('',#263468,#29346);
#24120=LINE('',#263544,#29347);
#24121=LINE('',#263620,#29348);
#24122=LINE('',#263696,#29349);
#24123=LINE('',#263772,#29350);
#24124=LINE('',#263850,#29351);
#24125=LINE('',#263920,#29352);
#24126=LINE('',#263930,#29353);
#24127=LINE('',#263994,#29354);
#24128=LINE('',#263996,#29355);
#24129=LINE('',#263998,#29356);
#24130=LINE('',#264000,#29357);
#24131=LINE('',#264002,#29358);
#24132=LINE('',#264003,#29359);
#24133=LINE('',#264005,#29360);
#24134=LINE('',#264006,#29361);
#24135=LINE('',#264008,#29362);
#24136=LINE('',#264010,#29363);
#24137=LINE('',#264012,#29364);
#24138=LINE('',#264014,#29365);
#24139=LINE('',#264699,#29366);
#24140=LINE('',#264707,#29367);
#24141=LINE('',#264713,#29368);
#24142=LINE('',#264721,#29369);
#24143=LINE('',#264725,#29370);
#24144=LINE('',#264745,#29371);
#24145=LINE('',#264806,#29372);
#24146=LINE('',#264843,#29373);
#24147=LINE('',#264883,#29374);
#24148=LINE('',#264884,#29375);
#24149=LINE('',#264891,#29376);
#24150=LINE('',#264897,#29377);
#24151=LINE('',#264910,#29378);
#24152=LINE('',#264916,#29379);
#24153=LINE('',#264919,#29380);
#24154=LINE('',#264924,#29381);
#24155=LINE('',#264930,#29382);
#24156=LINE('',#264936,#29383);
#24157=LINE('',#264942,#29384);
#24158=LINE('',#264948,#29385);
#24159=LINE('',#264954,#29386);
#24160=LINE('',#264960,#29387);
#24161=LINE('',#264966,#29388);
#24162=LINE('',#264972,#29389);
#24163=LINE('',#264978,#29390);
#24164=LINE('',#264983,#29391);
#24165=LINE('',#264987,#29392);
#24166=LINE('',#264991,#29393);
#24167=LINE('',#264993,#29394);
#24168=LINE('',#264994,#29395);
#24169=LINE('',#264999,#29396);
#24170=LINE('',#265003,#29397);
#24171=LINE('',#265005,#29398);
#24172=LINE('',#265006,#29399);
#24173=LINE('',#265011,#29400);
#24174=LINE('',#265015,#29401);
#24175=LINE('',#265017,#29402);
#24176=LINE('',#265018,#29403);
#24177=LINE('',#265023,#29404);
#24178=LINE('',#265026,#29405);
#24179=LINE('',#265027,#29406);
#24180=LINE('',#265031,#29407);
#24181=LINE('',#265035,#29408);
#24182=LINE('',#265039,#29409);
#24183=LINE('',#265043,#29410);
#24184=LINE('',#265054,#29411);
#24185=LINE('',#265058,#29412);
#24186=LINE('',#265062,#29413);
#24187=LINE('',#265065,#29414);
#24188=LINE('',#265068,#29415);
#24189=LINE('',#265071,#29416);
#24190=LINE('',#265074,#29417);
#24191=LINE('',#265075,#29418);
#24192=LINE('',#265078,#29419);
#24193=LINE('',#265082,#29420);
#24194=LINE('',#265083,#29421);
#24195=LINE('',#265086,#29422);
#24196=LINE('',#265090,#29423);
#24197=LINE('',#265091,#29424);
#24198=LINE('',#265094,#29425);
#24199=LINE('',#265097,#29426);
#24200=LINE('',#265118,#29427);
#24201=LINE('',#265122,#29428);
#24202=LINE('',#265126,#29429);
#24203=LINE('',#265129,#29430);
#24204=LINE('',#265131,#29431);
#24205=LINE('',#265134,#29432);
#24206=LINE('',#265140,#29433);
#24207=LINE('',#265143,#29434);
#24208=LINE('',#265145,#29435);
#24209=LINE('',#265147,#29436);
#24210=LINE('',#265150,#29437);
#24211=LINE('',#265153,#29438);
#24212=LINE('',#265155,#29439);
#24213=LINE('',#265156,#29440);
#25305=VECTOR('',#112081,1000.);
#25306=VECTOR('',#112082,1000.);
#25307=VECTOR('',#112091,5.1435);
#25308=VECTOR('',#112108,3.78554799125932);
#25309=VECTOR('',#112127,2.40973730802039);
#25310=VECTOR('',#112142,0.952499999999998);
#25311=VECTOR('',#112185,1000.);
#25312=VECTOR('',#112188,1000.);
#25313=VECTOR('',#112189,1000.);
#25314=VECTOR('',#112192,1000.);
#25315=VECTOR('',#112193,1000.);
#25316=VECTOR('',#112196,1000.);
#25317=VECTOR('',#112197,1000.);
#25318=VECTOR('',#112200,1000.);
#25319=VECTOR('',#112201,1000.);
#25320=VECTOR('',#112204,1000.);
#25321=VECTOR('',#112219,7.9375);
#25322=VECTOR('',#112226,8.4455);
#25323=VECTOR('',#112237,7.9375);
#25324=VECTOR('',#112244,8.4455);
#25325=VECTOR('',#112255,7.9375);
#25326=VECTOR('',#112262,8.4455);
#25327=VECTOR('',#112273,7.9375);
#25328=VECTOR('',#112280,8.4455);
#25329=VECTOR('',#112311,51.27);
#25330=VECTOR('',#112314,50.);
#25331=VECTOR('',#112345,56.875);
#25332=VECTOR('',#112348,55.605);
#25333=VECTOR('',#112359,51.27);
#25334=VECTOR('',#112366,55.605);
#25335=VECTOR('',#112455,65.);
#25336=VECTOR('',#112460,64.008019903844);
#25337=VECTOR('',#112465,10.);
#25338=VECTOR('',#112468,10.);
#25339=VECTOR('',#112471,10.);
#25340=VECTOR('',#112474,10.);
#25341=VECTOR('',#112477,10.);
#25342=VECTOR('',#112480,10.);
#25343=VECTOR('',#112483,10.);
#25344=VECTOR('',#112486,10.);
#25345=VECTOR('',#112489,10.);
#25346=VECTOR('',#112492,10.);
#25347=VECTOR('',#112495,10.);
#25348=VECTOR('',#112498,10.);
#25349=VECTOR('',#112501,10.);
#25350=VECTOR('',#112504,10.);
#25351=VECTOR('',#112507,10.);
#25352=VECTOR('',#112510,10.);
#25353=VECTOR('',#112513,10.);
#25354=VECTOR('',#112516,10.);
#25355=VECTOR('',#112519,10.);
#25356=VECTOR('',#112522,10.);
#25357=VECTOR('',#112525,10.);
#25358=VECTOR('',#112528,10.);
#25359=VECTOR('',#112531,10.);
#25360=VECTOR('',#112534,10.);
#25361=VECTOR('',#112537,10.);
#25362=VECTOR('',#112540,10.);
#25363=VECTOR('',#112543,10.);
#25364=VECTOR('',#112546,10.);
#25365=VECTOR('',#112549,10.);
#25366=VECTOR('',#112552,10.);
#25367=VECTOR('',#112555,10.);
#25368=VECTOR('',#112558,10.);
#25369=VECTOR('',#112561,10.);
#25370=VECTOR('',#112564,10.);
#25371=VECTOR('',#112567,10.);
#25372=VECTOR('',#112570,10.);
#25373=VECTOR('',#112573,10.);
#25374=VECTOR('',#112576,10.);
#25375=VECTOR('',#112579,10.);
#25376=VECTOR('',#112582,10.);
#25377=VECTOR('',#112585,10.);
#25378=VECTOR('',#112588,10.);
#25379=VECTOR('',#112591,10.);
#25380=VECTOR('',#112594,10.);
#25381=VECTOR('',#112597,10.);
#25382=VECTOR('',#112600,10.);
#25383=VECTOR('',#112603,10.);
#25384=VECTOR('',#112606,10.);
#25385=VECTOR('',#112609,10.);
#25386=VECTOR('',#112612,10.);
#25387=VECTOR('',#112615,10.);
#25388=VECTOR('',#112618,10.);
#25389=VECTOR('',#112621,10.);
#25390=VECTOR('',#112624,10.);
#25391=VECTOR('',#112627,10.);
#25392=VECTOR('',#112630,10.);
#25393=VECTOR('',#112633,10.);
#25394=VECTOR('',#112636,10.);
#25395=VECTOR('',#112639,10.);
#25396=VECTOR('',#112642,10.);
#25397=VECTOR('',#112643,62.2224557307631);
#25398=VECTOR('',#112644,10.);
#25399=VECTOR('',#112647,10.);
#25400=VECTOR('',#112650,10.);
#25401=VECTOR('',#112653,10.);
#25402=VECTOR('',#112656,10.);
#25403=VECTOR('',#112659,10.);
#25404=VECTOR('',#112662,10.);
#25405=VECTOR('',#112665,10.);
#25406=VECTOR('',#112668,10.);
#25407=VECTOR('',#112671,10.);
#25408=VECTOR('',#112674,10.);
#25409=VECTOR('',#112677,10.);
#25410=VECTOR('',#112680,10.);
#25411=VECTOR('',#112683,10.);
#25412=VECTOR('',#112686,10.);
#25413=VECTOR('',#112689,10.);
#25414=VECTOR('',#112692,10.);
#25415=VECTOR('',#112695,10.);
#25416=VECTOR('',#112698,10.);
#25417=VECTOR('',#112701,10.);
#25418=VECTOR('',#112704,10.);
#25419=VECTOR('',#112707,10.);
#25420=VECTOR('',#112710,10.);
#25421=VECTOR('',#112713,10.);
#25422=VECTOR('',#112716,10.);
#25423=VECTOR('',#112719,10.);
#25424=VECTOR('',#112722,10.);
#25425=VECTOR('',#112725,10.);
#25426=VECTOR('',#112728,10.);
#25427=VECTOR('',#112731,10.);
#25428=VECTOR('',#112732,10.);
#25429=VECTOR('',#112735,10.);
#25430=VECTOR('',#112738,10.);
#25431=VECTOR('',#112741,10.);
#25432=VECTOR('',#112744,10.);
#25433=VECTOR('',#112747,10.);
#25434=VECTOR('',#112750,10.);
#25435=VECTOR('',#112753,10.);
#25436=VECTOR('',#112756,10.);
#25437=VECTOR('',#112759,10.);
#25438=VECTOR('',#112762,10.);
#25439=VECTOR('',#112765,10.);
#25440=VECTOR('',#112768,10.);
#25441=VECTOR('',#112771,10.);
#25442=VECTOR('',#112774,10.);
#25443=VECTOR('',#112777,10.);
#25444=VECTOR('',#112780,10.);
#25445=VECTOR('',#112783,10.);
#25446=VECTOR('',#112786,10.);
#25447=VECTOR('',#112789,10.);
#25448=VECTOR('',#112792,10.);
#25449=VECTOR('',#112795,10.);
#25450=VECTOR('',#112798,10.);
#25451=VECTOR('',#112801,10.);
#25452=VECTOR('',#112804,10.);
#25453=VECTOR('',#112807,10.);
#25454=VECTOR('',#112810,10.);
#25455=VECTOR('',#112813,10.);
#25456=VECTOR('',#112816,10.);
#25457=VECTOR('',#112819,10.);
#25458=VECTOR('',#112822,10.);
#25459=VECTOR('',#112825,10.);
#25460=VECTOR('',#112828,10.);
#25461=VECTOR('',#112831,10.);
#25462=VECTOR('',#112834,10.);
#25463=VECTOR('',#112837,10.);
#25464=VECTOR('',#112840,10.);
#25465=VECTOR('',#112843,10.);
#25466=VECTOR('',#112846,10.);
#25467=VECTOR('',#112849,10.);
#25468=VECTOR('',#112852,10.);
#25469=VECTOR('',#112855,10.);
#25470=VECTOR('',#112858,10.);
#25471=VECTOR('',#112861,10.);
#25472=VECTOR('',#112864,10.);
#25473=VECTOR('',#112867,10.);
#25474=VECTOR('',#112870,10.);
#25475=VECTOR('',#112873,10.);
#25476=VECTOR('',#112876,10.);
#25477=VECTOR('',#112879,10.);
#25478=VECTOR('',#112882,10.);
#25479=VECTOR('',#112885,10.);
#25480=VECTOR('',#112888,10.);
#25481=VECTOR('',#112891,10.);
#25482=VECTOR('',#112894,10.);
#25483=VECTOR('',#112897,10.);
#25484=VECTOR('',#112900,10.);
#25485=VECTOR('',#112903,10.);
#25486=VECTOR('',#112906,10.);
#25487=VECTOR('',#112909,10.);
#25488=VECTOR('',#112912,10.);
#25489=VECTOR('',#112915,10.);
#25490=VECTOR('',#112918,10.);
#25491=VECTOR('',#112921,10.);
#25492=VECTOR('',#112924,10.);
#25493=VECTOR('',#112927,10.);
#25494=VECTOR('',#112930,10.);
#25495=VECTOR('',#112933,10.);
#25496=VECTOR('',#112936,10.);
#25497=VECTOR('',#112939,10.);
#25498=VECTOR('',#112942,10.);
#25499=VECTOR('',#112945,10.);
#25500=VECTOR('',#112948,10.);
#25501=VECTOR('',#112951,10.);
#25502=VECTOR('',#112954,10.);
#25503=VECTOR('',#112957,10.);
#25504=VECTOR('',#112960,10.);
#25505=VECTOR('',#112963,10.);
#25506=VECTOR('',#112966,10.);
#25507=VECTOR('',#112969,10.);
#25508=VECTOR('',#112972,10.);
#25509=VECTOR('',#112975,10.);
#25510=VECTOR('',#112978,10.);
#25511=VECTOR('',#112981,10.);
#25512=VECTOR('',#112984,10.);
#25513=VECTOR('',#112987,10.);
#25514=VECTOR('',#112990,10.);
#25515=VECTOR('',#112993,10.);
#25516=VECTOR('',#112996,10.);
#25517=VECTOR('',#112999,10.);
#25518=VECTOR('',#113002,58.6605641730809);
#25519=VECTOR('',#113005,10.);
#25520=VECTOR('',#113008,10.);
#25521=VECTOR('',#113011,10.);
#25522=VECTOR('',#113014,10.);
#25523=VECTOR('',#113017,10.);
#25524=VECTOR('',#113020,10.);
#25525=VECTOR('',#113023,10.);
#25526=VECTOR('',#113026,10.);
#25527=VECTOR('',#113029,10.);
#25528=VECTOR('',#113032,10.);
#25529=VECTOR('',#113035,10.);
#25530=VECTOR('',#113038,10.);
#25531=VECTOR('',#113041,10.);
#25532=VECTOR('',#113044,10.);
#25533=VECTOR('',#113047,10.);
#25534=VECTOR('',#113050,10.);
#25535=VECTOR('',#113053,10.);
#25536=VECTOR('',#113056,10.);
#25537=VECTOR('',#113059,10.);
#25538=VECTOR('',#113062,10.);
#25539=VECTOR('',#113065,10.);
#25540=VECTOR('',#113068,10.);
#25541=VECTOR('',#113071,10.);
#25542=VECTOR('',#113074,10.);
#25543=VECTOR('',#113077,10.);
#25544=VECTOR('',#113080,10.);
#25545=VECTOR('',#113083,10.);
#25546=VECTOR('',#113086,10.);
#25547=VECTOR('',#113089,10.);
#25548=VECTOR('',#113092,10.);
#25549=VECTOR('',#113093,10.);
#25550=VECTOR('',#113096,10.);
#25551=VECTOR('',#113099,10.);
#25552=VECTOR('',#113102,10.);
#25553=VECTOR('',#113105,10.);
#25554=VECTOR('',#113108,10.);
#25555=VECTOR('',#113111,10.);
#25556=VECTOR('',#113114,10.);
#25557=VECTOR('',#113117,10.);
#25558=VECTOR('',#113120,10.);
#25559=VECTOR('',#113123,10.);
#25560=VECTOR('',#113126,10.);
#25561=VECTOR('',#113129,10.);
#25562=VECTOR('',#113132,10.);
#25563=VECTOR('',#113135,10.);
#25564=VECTOR('',#113138,10.);
#25565=VECTOR('',#113141,10.);
#25566=VECTOR('',#113144,10.);
#25567=VECTOR('',#113147,10.);
#25568=VECTOR('',#113150,10.);
#25569=VECTOR('',#113153,10.);
#25570=VECTOR('',#113156,10.);
#25571=VECTOR('',#113159,10.);
#25572=VECTOR('',#113162,10.);
#25573=VECTOR('',#113165,10.);
#25574=VECTOR('',#113168,10.);
#25575=VECTOR('',#113171,10.);
#25576=VECTOR('',#113174,10.);
#25577=VECTOR('',#113177,10.);
#25578=VECTOR('',#113180,10.);
#25579=VECTOR('',#113185,56.875);
#25580=VECTOR('',#113190,56.875);
#25581=VECTOR('',#113197,1000.);
#25582=VECTOR('',#113200,1000.);
#25583=VECTOR('',#113209,10.);
#25584=VECTOR('',#113210,10.);
#25585=VECTOR('',#113215,1000.);
#25586=VECTOR('',#113218,1000.);
#25587=VECTOR('',#113223,10.);
#25588=VECTOR('',#113226,10.);
#25589=VECTOR('',#113235,1000.);
#25590=VECTOR('',#113236,1000.);
#25591=VECTOR('',#113265,1000.);
#25592=VECTOR('',#113272,1000.);
#25593=VECTOR('',#113275,10.);
#25594=VECTOR('',#113278,10.);
#25595=VECTOR('',#113283,1000.);
#25596=VECTOR('',#113286,1000.);
#25597=VECTOR('',#113291,10.);
#25598=VECTOR('',#113298,10.);
#25599=VECTOR('',#113301,1000.);
#25600=VECTOR('',#113304,1000.);
#25601=VECTOR('',#113333,1000.);
#25602=VECTOR('',#113340,1000.);
#25603=VECTOR('',#113343,10.);
#25604=VECTOR('',#113346,10.);
#25605=VECTOR('',#113351,1000.);
#25606=VECTOR('',#113354,1000.);
#25607=VECTOR('',#113359,10.);
#25608=VECTOR('',#113366,10.);
#25609=VECTOR('',#113369,1000.);
#25610=VECTOR('',#113372,1000.);
#25611=VECTOR('',#113401,1000.);
#25612=VECTOR('',#113408,1000.);
#25613=VECTOR('',#113411,10.);
#25614=VECTOR('',#113414,10.);
#25615=VECTOR('',#113419,1000.);
#25616=VECTOR('',#113422,1000.);
#25617=VECTOR('',#113427,10.);
#25618=VECTOR('',#113434,10.);
#25619=VECTOR('',#113437,1000.);
#25620=VECTOR('',#113440,1000.);
#25621=VECTOR('',#113469,1000.);
#25622=VECTOR('',#113476,1000.);
#25623=VECTOR('',#113479,10.);
#25624=VECTOR('',#113482,10.);
#25625=VECTOR('',#113487,1000.);
#25626=VECTOR('',#113490,1000.);
#25627=VECTOR('',#113495,10.);
#25628=VECTOR('',#113502,10.);
#25629=VECTOR('',#113505,1000.);
#25630=VECTOR('',#113508,1000.);
#25631=VECTOR('',#113537,1000.);
#25632=VECTOR('',#113544,1000.);
#25633=VECTOR('',#113547,10.);
#25634=VECTOR('',#113550,10.);
#25635=VECTOR('',#113555,1000.);
#25636=VECTOR('',#113558,1000.);
#25637=VECTOR('',#113563,10.);
#25638=VECTOR('',#113570,10.);
#25639=VECTOR('',#113573,1000.);
#25640=VECTOR('',#113576,1000.);
#25641=VECTOR('',#113605,1000.);
#25642=VECTOR('',#113612,1000.);
#25643=VECTOR('',#113615,10.);
#25644=VECTOR('',#113618,10.);
#25645=VECTOR('',#113623,1000.);
#25646=VECTOR('',#113626,1000.);
#25647=VECTOR('',#113631,10.);
#25648=VECTOR('',#113638,10.);
#25649=VECTOR('',#113641,1000.);
#25650=VECTOR('',#113644,1000.);
#25651=VECTOR('',#113673,1000.);
#25652=VECTOR('',#113680,1000.);
#25653=VECTOR('',#113683,10.);
#25654=VECTOR('',#113686,10.);
#25655=VECTOR('',#113691,1000.);
#25656=VECTOR('',#113694,1000.);
#25657=VECTOR('',#113699,10.);
#25658=VECTOR('',#113706,10.);
#25659=VECTOR('',#113709,1000.);
#25660=VECTOR('',#113712,1000.);
#25661=VECTOR('',#113741,1000.);
#25662=VECTOR('',#113748,1000.);
#25663=VECTOR('',#113751,10.);
#25664=VECTOR('',#113754,10.);
#25665=VECTOR('',#113759,1000.);
#25666=VECTOR('',#113762,1000.);
#25667=VECTOR('',#113767,10.);
#25668=VECTOR('',#113774,10.);
#25669=VECTOR('',#113777,1000.);
#25670=VECTOR('',#113780,1000.);
#25671=VECTOR('',#113809,1000.);
#25672=VECTOR('',#113816,1000.);
#25673=VECTOR('',#113819,10.);
#25674=VECTOR('',#113822,10.);
#25675=VECTOR('',#113827,1000.);
#25676=VECTOR('',#113830,1000.);
#25677=VECTOR('',#113835,10.);
#25678=VECTOR('',#113842,10.);
#25679=VECTOR('',#113845,1000.);
#25680=VECTOR('',#113848,1000.);
#25681=VECTOR('',#113877,1000.);
#25682=VECTOR('',#113884,1000.);
#25683=VECTOR('',#113887,10.);
#25684=VECTOR('',#113890,10.);
#25685=VECTOR('',#113895,1000.);
#25686=VECTOR('',#113898,1000.);
#25687=VECTOR('',#113903,10.);
#25688=VECTOR('',#113910,10.);
#25689=VECTOR('',#113913,1000.);
#25690=VECTOR('',#113916,1000.);
#25691=VECTOR('',#113945,1000.);
#25692=VECTOR('',#113952,1000.);
#25693=VECTOR('',#113955,10.);
#25694=VECTOR('',#113958,10.);
#25695=VECTOR('',#113963,1000.);
#25696=VECTOR('',#113966,1000.);
#25697=VECTOR('',#113971,10.);
#25698=VECTOR('',#113978,10.);
#25699=VECTOR('',#113981,1000.);
#25700=VECTOR('',#113984,1000.);
#25701=VECTOR('',#114013,1000.);
#25702=VECTOR('',#114020,1000.);
#25703=VECTOR('',#114023,10.);
#25704=VECTOR('',#114026,10.);
#25705=VECTOR('',#114031,1000.);
#25706=VECTOR('',#114034,1000.);
#25707=VECTOR('',#114039,10.);
#25708=VECTOR('',#114046,10.);
#25709=VECTOR('',#114049,1000.);
#25710=VECTOR('',#114052,1000.);
#25711=VECTOR('',#114081,1000.);
#25712=VECTOR('',#114088,1000.);
#25713=VECTOR('',#114091,10.);
#25714=VECTOR('',#114094,10.);
#25715=VECTOR('',#114099,1000.);
#25716=VECTOR('',#114102,1000.);
#25717=VECTOR('',#114107,10.);
#25718=VECTOR('',#114114,10.);
#25719=VECTOR('',#114117,1000.);
#25720=VECTOR('',#114120,1000.);
#25721=VECTOR('',#114149,1000.);
#25722=VECTOR('',#114156,1000.);
#25723=VECTOR('',#114159,10.);
#25724=VECTOR('',#114162,10.);
#25725=VECTOR('',#114167,1000.);
#25726=VECTOR('',#114170,1000.);
#25727=VECTOR('',#114175,10.);
#25728=VECTOR('',#114182,10.);
#25729=VECTOR('',#114185,1000.);
#25730=VECTOR('',#114188,1000.);
#25731=VECTOR('',#114217,1000.);
#25732=VECTOR('',#114224,1000.);
#25733=VECTOR('',#114227,10.);
#25734=VECTOR('',#114230,10.);
#25735=VECTOR('',#114235,1000.);
#25736=VECTOR('',#114238,1000.);
#25737=VECTOR('',#114243,10.);
#25738=VECTOR('',#114250,10.);
#25739=VECTOR('',#114253,1000.);
#25740=VECTOR('',#114256,1000.);
#25741=VECTOR('',#114285,1000.);
#25742=VECTOR('',#114292,1000.);
#25743=VECTOR('',#114295,10.);
#25744=VECTOR('',#114298,10.);
#25745=VECTOR('',#114303,1000.);
#25746=VECTOR('',#114306,1000.);
#25747=VECTOR('',#114311,10.);
#25748=VECTOR('',#114318,10.);
#25749=VECTOR('',#114321,1000.);
#25750=VECTOR('',#114324,1000.);
#25751=VECTOR('',#114353,1000.);
#25752=VECTOR('',#114360,1000.);
#25753=VECTOR('',#114363,10.);
#25754=VECTOR('',#114366,10.);
#25755=VECTOR('',#114371,1000.);
#25756=VECTOR('',#114374,1000.);
#25757=VECTOR('',#114379,10.);
#25758=VECTOR('',#114386,10.);
#25759=VECTOR('',#114389,1000.);
#25760=VECTOR('',#114392,1000.);
#25761=VECTOR('',#114421,1000.);
#25762=VECTOR('',#114428,1000.);
#25763=VECTOR('',#114431,10.);
#25764=VECTOR('',#114434,10.);
#25765=VECTOR('',#114439,1000.);
#25766=VECTOR('',#114442,1000.);
#25767=VECTOR('',#114447,10.);
#25768=VECTOR('',#114454,10.);
#25769=VECTOR('',#114457,1000.);
#25770=VECTOR('',#114460,1000.);
#25771=VECTOR('',#114489,1000.);
#25772=VECTOR('',#114496,1000.);
#25773=VECTOR('',#114499,10.);
#25774=VECTOR('',#114502,10.);
#25775=VECTOR('',#114507,1000.);
#25776=VECTOR('',#114510,1000.);
#25777=VECTOR('',#114515,10.);
#25778=VECTOR('',#114522,10.);
#25779=VECTOR('',#114525,1000.);
#25780=VECTOR('',#114528,1000.);
#25781=VECTOR('',#114557,1000.);
#25782=VECTOR('',#114564,1000.);
#25783=VECTOR('',#114567,10.);
#25784=VECTOR('',#114570,10.);
#25785=VECTOR('',#114575,1000.);
#25786=VECTOR('',#114578,1000.);
#25787=VECTOR('',#114583,10.);
#25788=VECTOR('',#114590,10.);
#25789=VECTOR('',#114593,1000.);
#25790=VECTOR('',#114596,1000.);
#25791=VECTOR('',#114625,1000.);
#25792=VECTOR('',#114632,1000.);
#25793=VECTOR('',#114635,10.);
#25794=VECTOR('',#114638,10.);
#25795=VECTOR('',#114643,1000.);
#25796=VECTOR('',#114646,1000.);
#25797=VECTOR('',#114651,10.);
#25798=VECTOR('',#114658,10.);
#25799=VECTOR('',#114661,1000.);
#25800=VECTOR('',#114664,1000.);
#25801=VECTOR('',#114693,1000.);
#25802=VECTOR('',#114700,1000.);
#25803=VECTOR('',#114703,10.);
#25804=VECTOR('',#114706,10.);
#25805=VECTOR('',#114711,1000.);
#25806=VECTOR('',#114714,1000.);
#25807=VECTOR('',#114719,10.);
#25808=VECTOR('',#114726,10.);
#25809=VECTOR('',#114729,1000.);
#25810=VECTOR('',#114732,1000.);
#25811=VECTOR('',#114761,1000.);
#25812=VECTOR('',#114768,1000.);
#25813=VECTOR('',#114771,10.);
#25814=VECTOR('',#114774,10.);
#25815=VECTOR('',#114779,1000.);
#25816=VECTOR('',#114782,1000.);
#25817=VECTOR('',#114787,10.);
#25818=VECTOR('',#114794,10.);
#25819=VECTOR('',#114797,1000.);
#25820=VECTOR('',#114800,1000.);
#25821=VECTOR('',#114829,1000.);
#25822=VECTOR('',#114836,1000.);
#25823=VECTOR('',#114839,10.);
#25824=VECTOR('',#114842,10.);
#25825=VECTOR('',#114847,1000.);
#25826=VECTOR('',#114850,1000.);
#25827=VECTOR('',#114855,10.);
#25828=VECTOR('',#114862,10.);
#25829=VECTOR('',#114865,1000.);
#25830=VECTOR('',#114868,1000.);
#25831=VECTOR('',#114897,1000.);
#25832=VECTOR('',#114904,1000.);
#25833=VECTOR('',#114907,10.);
#25834=VECTOR('',#114910,10.);
#25835=VECTOR('',#114915,1000.);
#25836=VECTOR('',#114918,1000.);
#25837=VECTOR('',#114923,10.);
#25838=VECTOR('',#114930,10.);
#25839=VECTOR('',#114933,1000.);
#25840=VECTOR('',#114936,1000.);
#25841=VECTOR('',#114965,1000.);
#25842=VECTOR('',#114972,1000.);
#25843=VECTOR('',#114975,10.);
#25844=VECTOR('',#114978,10.);
#25845=VECTOR('',#114983,1000.);
#25846=VECTOR('',#114986,1000.);
#25847=VECTOR('',#114991,10.);
#25848=VECTOR('',#114998,10.);
#25849=VECTOR('',#115001,1000.);
#25850=VECTOR('',#115004,1000.);
#25851=VECTOR('',#115033,1000.);
#25852=VECTOR('',#115040,1000.);
#25853=VECTOR('',#115043,10.);
#25854=VECTOR('',#115046,10.);
#25855=VECTOR('',#115051,1000.);
#25856=VECTOR('',#115054,1000.);
#25857=VECTOR('',#115059,10.);
#25858=VECTOR('',#115066,10.);
#25859=VECTOR('',#115069,1000.);
#25860=VECTOR('',#115072,1000.);
#25861=VECTOR('',#115101,1000.);
#25862=VECTOR('',#115108,1000.);
#25863=VECTOR('',#115111,10.);
#25864=VECTOR('',#115114,10.);
#25865=VECTOR('',#115119,1000.);
#25866=VECTOR('',#115122,1000.);
#25867=VECTOR('',#115127,10.);
#25868=VECTOR('',#115134,10.);
#25869=VECTOR('',#115137,1000.);
#25870=VECTOR('',#115140,1000.);
#25871=VECTOR('',#115169,1000.);
#25872=VECTOR('',#115176,1000.);
#25873=VECTOR('',#115179,10.);
#25874=VECTOR('',#115182,10.);
#25875=VECTOR('',#115187,1000.);
#25876=VECTOR('',#115190,1000.);
#25877=VECTOR('',#115195,10.);
#25878=VECTOR('',#115202,10.);
#25879=VECTOR('',#115205,1000.);
#25880=VECTOR('',#115208,1000.);
#25881=VECTOR('',#115237,1000.);
#25882=VECTOR('',#115244,1000.);
#25883=VECTOR('',#115247,10.);
#25884=VECTOR('',#115250,10.);
#25885=VECTOR('',#115255,1000.);
#25886=VECTOR('',#115258,1000.);
#25887=VECTOR('',#115263,10.);
#25888=VECTOR('',#115270,10.);
#25889=VECTOR('',#115273,1000.);
#25890=VECTOR('',#115276,1000.);
#25891=VECTOR('',#115305,1000.);
#25892=VECTOR('',#115312,1000.);
#25893=VECTOR('',#115315,10.);
#25894=VECTOR('',#115318,10.);
#25895=VECTOR('',#115323,1000.);
#25896=VECTOR('',#115326,1000.);
#25897=VECTOR('',#115331,10.);
#25898=VECTOR('',#115338,10.);
#25899=VECTOR('',#115341,1000.);
#25900=VECTOR('',#115344,1000.);
#25901=VECTOR('',#115373,1000.);
#25902=VECTOR('',#115380,1000.);
#25903=VECTOR('',#115383,10.);
#25904=VECTOR('',#115386,10.);
#25905=VECTOR('',#115391,1000.);
#25906=VECTOR('',#115394,1000.);
#25907=VECTOR('',#115399,10.);
#25908=VECTOR('',#115406,10.);
#25909=VECTOR('',#115409,1000.);
#25910=VECTOR('',#115412,1000.);
#25911=VECTOR('',#115441,1000.);
#25912=VECTOR('',#115448,1000.);
#25913=VECTOR('',#115451,10.);
#25914=VECTOR('',#115454,10.);
#25915=VECTOR('',#115459,1000.);
#25916=VECTOR('',#115462,1000.);
#25917=VECTOR('',#115467,10.);
#25918=VECTOR('',#115474,10.);
#25919=VECTOR('',#115477,1000.);
#25920=VECTOR('',#115480,1000.);
#25921=VECTOR('',#115509,1000.);
#25922=VECTOR('',#115516,1000.);
#25923=VECTOR('',#115519,10.);
#25924=VECTOR('',#115522,10.);
#25925=VECTOR('',#115527,1000.);
#25926=VECTOR('',#115530,1000.);
#25927=VECTOR('',#115535,10.);
#25928=VECTOR('',#115542,10.);
#25929=VECTOR('',#115545,1000.);
#25930=VECTOR('',#115548,1000.);
#25931=VECTOR('',#115577,1000.);
#25932=VECTOR('',#115584,1000.);
#25933=VECTOR('',#115587,10.);
#25934=VECTOR('',#115590,10.);
#25935=VECTOR('',#115595,1000.);
#25936=VECTOR('',#115598,1000.);
#25937=VECTOR('',#115603,10.);
#25938=VECTOR('',#115610,10.);
#25939=VECTOR('',#115613,1000.);
#25940=VECTOR('',#115616,1000.);
#25941=VECTOR('',#115645,1000.);
#25942=VECTOR('',#115652,1000.);
#25943=VECTOR('',#115655,10.);
#25944=VECTOR('',#115658,10.);
#25945=VECTOR('',#115663,1000.);
#25946=VECTOR('',#115666,1000.);
#25947=VECTOR('',#115671,10.);
#25948=VECTOR('',#115678,10.);
#25949=VECTOR('',#115681,1000.);
#25950=VECTOR('',#115684,1000.);
#25951=VECTOR('',#115713,1000.);
#25952=VECTOR('',#115720,1000.);
#25953=VECTOR('',#115723,10.);
#25954=VECTOR('',#115726,10.);
#25955=VECTOR('',#115731,1000.);
#25956=VECTOR('',#115734,1000.);
#25957=VECTOR('',#115739,10.);
#25958=VECTOR('',#115746,10.);
#25959=VECTOR('',#115749,1000.);
#25960=VECTOR('',#115752,1000.);
#25961=VECTOR('',#115781,1000.);
#25962=VECTOR('',#115788,1000.);
#25963=VECTOR('',#115791,10.);
#25964=VECTOR('',#115794,10.);
#25965=VECTOR('',#115799,1000.);
#25966=VECTOR('',#115802,1000.);
#25967=VECTOR('',#115807,10.);
#25968=VECTOR('',#115814,10.);
#25969=VECTOR('',#115817,1000.);
#25970=VECTOR('',#115820,1000.);
#25971=VECTOR('',#115849,1000.);
#25972=VECTOR('',#115856,1000.);
#25973=VECTOR('',#115859,10.);
#25974=VECTOR('',#115862,10.);
#25975=VECTOR('',#115867,1000.);
#25976=VECTOR('',#115870,1000.);
#25977=VECTOR('',#115875,10.);
#25978=VECTOR('',#115882,10.);
#25979=VECTOR('',#115885,1000.);
#25980=VECTOR('',#115888,1000.);
#25981=VECTOR('',#115917,1000.);
#25982=VECTOR('',#115924,1000.);
#25983=VECTOR('',#115927,10.);
#25984=VECTOR('',#115930,10.);
#25985=VECTOR('',#115935,1000.);
#25986=VECTOR('',#115938,1000.);
#25987=VECTOR('',#115943,10.);
#25988=VECTOR('',#115950,10.);
#25989=VECTOR('',#115953,1000.);
#25990=VECTOR('',#115956,1000.);
#25991=VECTOR('',#115985,1000.);
#25992=VECTOR('',#115992,1000.);
#25993=VECTOR('',#115995,10.);
#25994=VECTOR('',#115998,10.);
#25995=VECTOR('',#116003,1000.);
#25996=VECTOR('',#116006,1000.);
#25997=VECTOR('',#116011,10.);
#25998=VECTOR('',#116018,10.);
#25999=VECTOR('',#116021,1000.);
#26000=VECTOR('',#116024,1000.);
#26001=VECTOR('',#116053,1000.);
#26002=VECTOR('',#116060,1000.);
#26003=VECTOR('',#116063,10.);
#26004=VECTOR('',#116066,10.);
#26005=VECTOR('',#116071,1000.);
#26006=VECTOR('',#116074,1000.);
#26007=VECTOR('',#116079,10.);
#26008=VECTOR('',#116086,10.);
#26009=VECTOR('',#116089,1000.);
#26010=VECTOR('',#116092,1000.);
#26011=VECTOR('',#116121,1000.);
#26012=VECTOR('',#116128,1000.);
#26013=VECTOR('',#116131,10.);
#26014=VECTOR('',#116134,10.);
#26015=VECTOR('',#116139,1000.);
#26016=VECTOR('',#116142,1000.);
#26017=VECTOR('',#116147,10.);
#26018=VECTOR('',#116154,10.);
#26019=VECTOR('',#116157,1000.);
#26020=VECTOR('',#116160,1000.);
#26021=VECTOR('',#116189,1000.);
#26022=VECTOR('',#116196,1000.);
#26023=VECTOR('',#116199,10.);
#26024=VECTOR('',#116202,10.);
#26025=VECTOR('',#116207,1000.);
#26026=VECTOR('',#116210,1000.);
#26027=VECTOR('',#116215,10.);
#26028=VECTOR('',#116222,10.);
#26029=VECTOR('',#116225,1000.);
#26030=VECTOR('',#116228,1000.);
#26031=VECTOR('',#116257,1000.);
#26032=VECTOR('',#116264,1000.);
#26033=VECTOR('',#116267,10.);
#26034=VECTOR('',#116270,10.);
#26035=VECTOR('',#116275,1000.);
#26036=VECTOR('',#116278,1000.);
#26037=VECTOR('',#116283,10.);
#26038=VECTOR('',#116290,10.);
#26039=VECTOR('',#116293,1000.);
#26040=VECTOR('',#116296,1000.);
#26041=VECTOR('',#116325,1000.);
#26042=VECTOR('',#116332,1000.);
#26043=VECTOR('',#116335,10.);
#26044=VECTOR('',#116338,10.);
#26045=VECTOR('',#116343,1000.);
#26046=VECTOR('',#116346,1000.);
#26047=VECTOR('',#116351,10.);
#26048=VECTOR('',#116358,10.);
#26049=VECTOR('',#116361,1000.);
#26050=VECTOR('',#116364,1000.);
#26051=VECTOR('',#116393,1000.);
#26052=VECTOR('',#116400,1000.);
#26053=VECTOR('',#116403,10.);
#26054=VECTOR('',#116406,10.);
#26055=VECTOR('',#116411,1000.);
#26056=VECTOR('',#116414,1000.);
#26057=VECTOR('',#116419,10.);
#26058=VECTOR('',#116426,10.);
#26059=VECTOR('',#116429,1000.);
#26060=VECTOR('',#116432,1000.);
#26061=VECTOR('',#116461,1000.);
#26062=VECTOR('',#116468,1000.);
#26063=VECTOR('',#116471,10.);
#26064=VECTOR('',#116474,10.);
#26065=VECTOR('',#116479,1000.);
#26066=VECTOR('',#116482,1000.);
#26067=VECTOR('',#116487,10.);
#26068=VECTOR('',#116494,10.);
#26069=VECTOR('',#116497,1000.);
#26070=VECTOR('',#116500,1000.);
#26071=VECTOR('',#116529,1000.);
#26072=VECTOR('',#116536,1000.);
#26073=VECTOR('',#116539,10.);
#26074=VECTOR('',#116542,10.);
#26075=VECTOR('',#116547,1000.);
#26076=VECTOR('',#116550,1000.);
#26077=VECTOR('',#116555,10.);
#26078=VECTOR('',#116562,10.);
#26079=VECTOR('',#116565,1000.);
#26080=VECTOR('',#116568,1000.);
#26081=VECTOR('',#116597,1000.);
#26082=VECTOR('',#116604,1000.);
#26083=VECTOR('',#116607,10.);
#26084=VECTOR('',#116610,10.);
#26085=VECTOR('',#116615,1000.);
#26086=VECTOR('',#116618,1000.);
#26087=VECTOR('',#116623,10.);
#26088=VECTOR('',#116630,10.);
#26089=VECTOR('',#116633,1000.);
#26090=VECTOR('',#116636,1000.);
#26091=VECTOR('',#116665,1000.);
#26092=VECTOR('',#116672,1000.);
#26093=VECTOR('',#116675,10.);
#26094=VECTOR('',#116678,10.);
#26095=VECTOR('',#116683,1000.);
#26096=VECTOR('',#116686,1000.);
#26097=VECTOR('',#116691,10.);
#26098=VECTOR('',#116698,10.);
#26099=VECTOR('',#116701,1000.);
#26100=VECTOR('',#116704,1000.);
#26101=VECTOR('',#116733,1000.);
#26102=VECTOR('',#116740,1000.);
#26103=VECTOR('',#116743,10.);
#26104=VECTOR('',#116746,10.);
#26105=VECTOR('',#116751,1000.);
#26106=VECTOR('',#116754,1000.);
#26107=VECTOR('',#116759,10.);
#26108=VECTOR('',#116766,10.);
#26109=VECTOR('',#116769,1000.);
#26110=VECTOR('',#116772,1000.);
#26111=VECTOR('',#116801,1000.);
#26112=VECTOR('',#116808,1000.);
#26113=VECTOR('',#116811,10.);
#26114=VECTOR('',#116814,10.);
#26115=VECTOR('',#116819,1000.);
#26116=VECTOR('',#116822,1000.);
#26117=VECTOR('',#116827,10.);
#26118=VECTOR('',#116834,10.);
#26119=VECTOR('',#116837,1000.);
#26120=VECTOR('',#116840,1000.);
#26121=VECTOR('',#116869,1000.);
#26122=VECTOR('',#116876,1000.);
#26123=VECTOR('',#116879,10.);
#26124=VECTOR('',#116882,10.);
#26125=VECTOR('',#116887,1000.);
#26126=VECTOR('',#116890,1000.);
#26127=VECTOR('',#116895,10.);
#26128=VECTOR('',#116902,10.);
#26129=VECTOR('',#116905,1000.);
#26130=VECTOR('',#116908,1000.);
#26131=VECTOR('',#116937,1000.);
#26132=VECTOR('',#116944,1000.);
#26133=VECTOR('',#116947,10.);
#26134=VECTOR('',#116950,10.);
#26135=VECTOR('',#116955,1000.);
#26136=VECTOR('',#116958,1000.);
#26137=VECTOR('',#116963,10.);
#26138=VECTOR('',#116970,10.);
#26139=VECTOR('',#116973,1000.);
#26140=VECTOR('',#116976,1000.);
#26141=VECTOR('',#117005,1000.);
#26142=VECTOR('',#117012,1000.);
#26143=VECTOR('',#117015,10.);
#26144=VECTOR('',#117018,10.);
#26145=VECTOR('',#117023,1000.);
#26146=VECTOR('',#117026,1000.);
#26147=VECTOR('',#117031,10.);
#26148=VECTOR('',#117038,10.);
#26149=VECTOR('',#117041,1000.);
#26150=VECTOR('',#117044,1000.);
#26151=VECTOR('',#117073,1000.);
#26152=VECTOR('',#117080,1000.);
#26153=VECTOR('',#117083,10.);
#26154=VECTOR('',#117086,10.);
#26155=VECTOR('',#117091,1000.);
#26156=VECTOR('',#117094,1000.);
#26157=VECTOR('',#117099,10.);
#26158=VECTOR('',#117106,10.);
#26159=VECTOR('',#117109,1000.);
#26160=VECTOR('',#117112,1000.);
#26161=VECTOR('',#117141,1000.);
#26162=VECTOR('',#117148,1000.);
#26163=VECTOR('',#117151,10.);
#26164=VECTOR('',#117154,10.);
#26165=VECTOR('',#117159,1000.);
#26166=VECTOR('',#117162,1000.);
#26167=VECTOR('',#117167,10.);
#26168=VECTOR('',#117174,10.);
#26169=VECTOR('',#117177,1000.);
#26170=VECTOR('',#117180,1000.);
#26171=VECTOR('',#117211,1000.);
#26172=VECTOR('',#117218,1000.);
#26173=VECTOR('',#117221,10.);
#26174=VECTOR('',#117224,10.);
#26175=VECTOR('',#117229,1000.);
#26176=VECTOR('',#117232,1000.);
#26177=VECTOR('',#117237,10.);
#26178=VECTOR('',#117244,10.);
#26179=VECTOR('',#117247,1000.);
#26180=VECTOR('',#117250,1000.);
#26181=VECTOR('',#117281,1000.);
#26182=VECTOR('',#117284,1000.);
#26183=VECTOR('',#117291,10.);
#26184=VECTOR('',#117292,1000.);
#26185=VECTOR('',#117293,10.);
#26186=VECTOR('',#117296,1000.);
#26187=VECTOR('',#117297,10.);
#26188=VECTOR('',#117300,1000.);
#26189=VECTOR('',#117303,10.);
#26190=VECTOR('',#117304,1000.);
#26191=VECTOR('',#117309,10.);
#26192=VECTOR('',#117310,1000.);
#26193=VECTOR('',#117311,10.);
#26194=VECTOR('',#117314,1000.);
#26195=VECTOR('',#117315,10.);
#26196=VECTOR('',#117318,1000.);
#26197=VECTOR('',#117321,10.);
#26198=VECTOR('',#117322,1000.);
#26199=VECTOR('',#117417,1000.);
#26200=VECTOR('',#117420,1000.);
#26201=VECTOR('',#117427,10.);
#26202=VECTOR('',#117428,1000.);
#26203=VECTOR('',#117429,10.);
#26204=VECTOR('',#117432,1000.);
#26205=VECTOR('',#117433,10.);
#26206=VECTOR('',#117436,1000.);
#26207=VECTOR('',#117439,10.);
#26208=VECTOR('',#117440,1000.);
#26209=VECTOR('',#117445,10.);
#26210=VECTOR('',#117446,1000.);
#26211=VECTOR('',#117447,10.);
#26212=VECTOR('',#117450,1000.);
#26213=VECTOR('',#117451,10.);
#26214=VECTOR('',#117454,1000.);
#26215=VECTOR('',#117457,10.);
#26216=VECTOR('',#117458,1000.);
#26217=VECTOR('',#117461,1000.);
#26218=VECTOR('',#117464,1000.);
#26219=VECTOR('',#117471,10.);
#26220=VECTOR('',#117472,1000.);
#26221=VECTOR('',#117473,10.);
#26222=VECTOR('',#117476,1000.);
#26223=VECTOR('',#117477,10.);
#26224=VECTOR('',#117480,1000.);
#26225=VECTOR('',#117483,10.);
#26226=VECTOR('',#117484,1000.);
#26227=VECTOR('',#117489,10.);
#26228=VECTOR('',#117490,1000.);
#26229=VECTOR('',#117491,10.);
#26230=VECTOR('',#117494,1000.);
#26231=VECTOR('',#117495,10.);
#26232=VECTOR('',#117498,1000.);
#26233=VECTOR('',#117501,10.);
#26234=VECTOR('',#117502,1000.);
#26235=VECTOR('',#117505,1000.);
#26236=VECTOR('',#117508,1000.);
#26237=VECTOR('',#117515,10.);
#26238=VECTOR('',#117516,1000.);
#26239=VECTOR('',#117517,10.);
#26240=VECTOR('',#117520,1000.);
#26241=VECTOR('',#117521,10.);
#26242=VECTOR('',#117524,1000.);
#26243=VECTOR('',#117527,10.);
#26244=VECTOR('',#117528,1000.);
#26245=VECTOR('',#117533,10.);
#26246=VECTOR('',#117534,1000.);
#26247=VECTOR('',#117535,10.);
#26248=VECTOR('',#117538,1000.);
#26249=VECTOR('',#117539,10.);
#26250=VECTOR('',#117542,1000.);
#26251=VECTOR('',#117545,10.);
#26252=VECTOR('',#117546,1000.);
#26253=VECTOR('',#117549,1000.);
#26254=VECTOR('',#117552,1000.);
#26255=VECTOR('',#117559,10.);
#26256=VECTOR('',#117560,1000.);
#26257=VECTOR('',#117561,10.);
#26258=VECTOR('',#117564,1000.);
#26259=VECTOR('',#117565,10.);
#26260=VECTOR('',#117568,1000.);
#26261=VECTOR('',#117571,10.);
#26262=VECTOR('',#117572,1000.);
#26263=VECTOR('',#117577,10.);
#26264=VECTOR('',#117578,1000.);
#26265=VECTOR('',#117579,10.);
#26266=VECTOR('',#117582,1000.);
#26267=VECTOR('',#117583,10.);
#26268=VECTOR('',#117586,1000.);
#26269=VECTOR('',#117589,10.);
#26270=VECTOR('',#117590,1000.);
#26271=VECTOR('',#117593,1000.);
#26272=VECTOR('',#117596,1000.);
#26273=VECTOR('',#117603,10.);
#26274=VECTOR('',#117604,1000.);
#26275=VECTOR('',#117605,10.);
#26276=VECTOR('',#117608,1000.);
#26277=VECTOR('',#117609,10.);
#26278=VECTOR('',#117612,1000.);
#26279=VECTOR('',#117615,10.);
#26280=VECTOR('',#117616,1000.);
#26281=VECTOR('',#117621,10.);
#26282=VECTOR('',#117622,1000.);
#26283=VECTOR('',#117623,10.);
#26284=VECTOR('',#117626,1000.);
#26285=VECTOR('',#117627,10.);
#26286=VECTOR('',#117630,1000.);
#26287=VECTOR('',#117633,10.);
#26288=VECTOR('',#117634,1000.);
#26289=VECTOR('',#117637,1000.);
#26290=VECTOR('',#117640,1000.);
#26291=VECTOR('',#117647,10.);
#26292=VECTOR('',#117648,1000.);
#26293=VECTOR('',#117649,10.);
#26294=VECTOR('',#117652,1000.);
#26295=VECTOR('',#117653,10.);
#26296=VECTOR('',#117656,1000.);
#26297=VECTOR('',#117659,10.);
#26298=VECTOR('',#117660,1000.);
#26299=VECTOR('',#117665,10.);
#26300=VECTOR('',#117666,1000.);
#26301=VECTOR('',#117667,10.);
#26302=VECTOR('',#117670,1000.);
#26303=VECTOR('',#117671,10.);
#26304=VECTOR('',#117674,1000.);
#26305=VECTOR('',#117677,10.);
#26306=VECTOR('',#117678,1000.);
#26307=VECTOR('',#117681,1000.);
#26308=VECTOR('',#117684,1000.);
#26309=VECTOR('',#117691,10.);
#26310=VECTOR('',#117692,1000.);
#26311=VECTOR('',#117693,10.);
#26312=VECTOR('',#117696,1000.);
#26313=VECTOR('',#117697,10.);
#26314=VECTOR('',#117700,1000.);
#26315=VECTOR('',#117703,10.);
#26316=VECTOR('',#117704,1000.);
#26317=VECTOR('',#117709,10.);
#26318=VECTOR('',#117710,1000.);
#26319=VECTOR('',#117711,10.);
#26320=VECTOR('',#117714,1000.);
#26321=VECTOR('',#117715,10.);
#26322=VECTOR('',#117718,1000.);
#26323=VECTOR('',#117721,10.);
#26324=VECTOR('',#117722,1000.);
#26325=VECTOR('',#117725,1000.);
#26326=VECTOR('',#117728,1000.);
#26327=VECTOR('',#117735,10.);
#26328=VECTOR('',#117736,1000.);
#26329=VECTOR('',#117737,10.);
#26330=VECTOR('',#117740,1000.);
#26331=VECTOR('',#117741,10.);
#26332=VECTOR('',#117744,1000.);
#26333=VECTOR('',#117747,10.);
#26334=VECTOR('',#117748,1000.);
#26335=VECTOR('',#117753,10.);
#26336=VECTOR('',#117754,1000.);
#26337=VECTOR('',#117755,10.);
#26338=VECTOR('',#117758,1000.);
#26339=VECTOR('',#117759,10.);
#26340=VECTOR('',#117762,1000.);
#26341=VECTOR('',#117765,10.);
#26342=VECTOR('',#117766,1000.);
#26343=VECTOR('',#117769,1000.);
#26344=VECTOR('',#117772,1000.);
#26345=VECTOR('',#117779,10.);
#26346=VECTOR('',#117780,1000.);
#26347=VECTOR('',#117781,10.);
#26348=VECTOR('',#117784,1000.);
#26349=VECTOR('',#117785,10.);
#26350=VECTOR('',#117788,1000.);
#26351=VECTOR('',#117791,10.);
#26352=VECTOR('',#117792,1000.);
#26353=VECTOR('',#117797,10.);
#26354=VECTOR('',#117798,1000.);
#26355=VECTOR('',#117799,10.);
#26356=VECTOR('',#117802,1000.);
#26357=VECTOR('',#117803,10.);
#26358=VECTOR('',#117806,1000.);
#26359=VECTOR('',#117809,10.);
#26360=VECTOR('',#117810,1000.);
#26361=VECTOR('',#117813,1000.);
#26362=VECTOR('',#117816,1000.);
#26363=VECTOR('',#117823,10.);
#26364=VECTOR('',#117824,1000.);
#26365=VECTOR('',#117825,10.);
#26366=VECTOR('',#117828,1000.);
#26367=VECTOR('',#117829,10.);
#26368=VECTOR('',#117832,1000.);
#26369=VECTOR('',#117835,10.);
#26370=VECTOR('',#117836,1000.);
#26371=VECTOR('',#117841,10.);
#26372=VECTOR('',#117842,1000.);
#26373=VECTOR('',#117843,10.);
#26374=VECTOR('',#117846,1000.);
#26375=VECTOR('',#117847,10.);
#26376=VECTOR('',#117850,1000.);
#26377=VECTOR('',#117853,10.);
#26378=VECTOR('',#117854,1000.);
#26379=VECTOR('',#117857,1000.);
#26380=VECTOR('',#117860,1000.);
#26381=VECTOR('',#117867,10.);
#26382=VECTOR('',#117868,1000.);
#26383=VECTOR('',#117869,10.);
#26384=VECTOR('',#117872,1000.);
#26385=VECTOR('',#117873,10.);
#26386=VECTOR('',#117876,1000.);
#26387=VECTOR('',#117879,10.);
#26388=VECTOR('',#117880,1000.);
#26389=VECTOR('',#117885,10.);
#26390=VECTOR('',#117886,1000.);
#26391=VECTOR('',#117887,10.);
#26392=VECTOR('',#117890,1000.);
#26393=VECTOR('',#117891,10.);
#26394=VECTOR('',#117894,1000.);
#26395=VECTOR('',#117897,10.);
#26396=VECTOR('',#117898,1000.);
#26397=VECTOR('',#117901,1000.);
#26398=VECTOR('',#117904,1000.);
#26399=VECTOR('',#117911,10.);
#26400=VECTOR('',#117912,1000.);
#26401=VECTOR('',#117913,10.);
#26402=VECTOR('',#117916,1000.);
#26403=VECTOR('',#117917,10.);
#26404=VECTOR('',#117920,1000.);
#26405=VECTOR('',#117923,10.);
#26406=VECTOR('',#117924,1000.);
#26407=VECTOR('',#117929,10.);
#26408=VECTOR('',#117930,1000.);
#26409=VECTOR('',#117931,10.);
#26410=VECTOR('',#117934,1000.);
#26411=VECTOR('',#117935,10.);
#26412=VECTOR('',#117938,1000.);
#26413=VECTOR('',#117941,10.);
#26414=VECTOR('',#117942,1000.);
#26415=VECTOR('',#117945,1000.);
#26416=VECTOR('',#117948,1000.);
#26417=VECTOR('',#117955,10.);
#26418=VECTOR('',#117956,1000.);
#26419=VECTOR('',#117957,10.);
#26420=VECTOR('',#117960,1000.);
#26421=VECTOR('',#117961,10.);
#26422=VECTOR('',#117964,1000.);
#26423=VECTOR('',#117967,10.);
#26424=VECTOR('',#117968,1000.);
#26425=VECTOR('',#117973,10.);
#26426=VECTOR('',#117974,1000.);
#26427=VECTOR('',#117975,10.);
#26428=VECTOR('',#117978,1000.);
#26429=VECTOR('',#117979,10.);
#26430=VECTOR('',#117982,1000.);
#26431=VECTOR('',#117985,10.);
#26432=VECTOR('',#117986,1000.);
#26433=VECTOR('',#117989,1000.);
#26434=VECTOR('',#117992,1000.);
#26435=VECTOR('',#117999,10.);
#26436=VECTOR('',#118000,1000.);
#26437=VECTOR('',#118001,10.);
#26438=VECTOR('',#118004,1000.);
#26439=VECTOR('',#118005,10.);
#26440=VECTOR('',#118008,1000.);
#26441=VECTOR('',#118011,10.);
#26442=VECTOR('',#118012,1000.);
#26443=VECTOR('',#118017,10.);
#26444=VECTOR('',#118018,1000.);
#26445=VECTOR('',#118019,10.);
#26446=VECTOR('',#118022,1000.);
#26447=VECTOR('',#118023,10.);
#26448=VECTOR('',#118026,1000.);
#26449=VECTOR('',#118029,10.);
#26450=VECTOR('',#118030,1000.);
#26451=VECTOR('',#118033,1000.);
#26452=VECTOR('',#118036,1000.);
#26453=VECTOR('',#118043,10.);
#26454=VECTOR('',#118044,1000.);
#26455=VECTOR('',#118045,10.);
#26456=VECTOR('',#118048,1000.);
#26457=VECTOR('',#118049,10.);
#26458=VECTOR('',#118052,1000.);
#26459=VECTOR('',#118055,10.);
#26460=VECTOR('',#118056,1000.);
#26461=VECTOR('',#118061,10.);
#26462=VECTOR('',#118062,1000.);
#26463=VECTOR('',#118063,10.);
#26464=VECTOR('',#118066,1000.);
#26465=VECTOR('',#118067,10.);
#26466=VECTOR('',#118070,1000.);
#26467=VECTOR('',#118073,10.);
#26468=VECTOR('',#118074,1000.);
#26469=VECTOR('',#118077,1000.);
#26470=VECTOR('',#118080,1000.);
#26471=VECTOR('',#118087,10.);
#26472=VECTOR('',#118088,1000.);
#26473=VECTOR('',#118089,10.);
#26474=VECTOR('',#118092,1000.);
#26475=VECTOR('',#118093,10.);
#26476=VECTOR('',#118096,1000.);
#26477=VECTOR('',#118099,10.);
#26478=VECTOR('',#118100,1000.);
#26479=VECTOR('',#118105,10.);
#26480=VECTOR('',#118106,1000.);
#26481=VECTOR('',#118107,10.);
#26482=VECTOR('',#118110,1000.);
#26483=VECTOR('',#118111,10.);
#26484=VECTOR('',#118114,1000.);
#26485=VECTOR('',#118117,10.);
#26486=VECTOR('',#118118,1000.);
#26487=VECTOR('',#118121,1000.);
#26488=VECTOR('',#118124,1000.);
#26489=VECTOR('',#118131,10.);
#26490=VECTOR('',#118132,1000.);
#26491=VECTOR('',#118133,10.);
#26492=VECTOR('',#118136,1000.);
#26493=VECTOR('',#118137,10.);
#26494=VECTOR('',#118140,1000.);
#26495=VECTOR('',#118143,10.);
#26496=VECTOR('',#118144,1000.);
#26497=VECTOR('',#118149,10.);
#26498=VECTOR('',#118150,1000.);
#26499=VECTOR('',#118151,10.);
#26500=VECTOR('',#118154,1000.);
#26501=VECTOR('',#118155,10.);
#26502=VECTOR('',#118158,1000.);
#26503=VECTOR('',#118161,10.);
#26504=VECTOR('',#118162,1000.);
#26505=VECTOR('',#118165,1000.);
#26506=VECTOR('',#118168,1000.);
#26507=VECTOR('',#118175,10.);
#26508=VECTOR('',#118176,1000.);
#26509=VECTOR('',#118177,10.);
#26510=VECTOR('',#118180,1000.);
#26511=VECTOR('',#118181,10.);
#26512=VECTOR('',#118184,1000.);
#26513=VECTOR('',#118187,10.);
#26514=VECTOR('',#118188,1000.);
#26515=VECTOR('',#118193,10.);
#26516=VECTOR('',#118194,1000.);
#26517=VECTOR('',#118195,10.);
#26518=VECTOR('',#118198,1000.);
#26519=VECTOR('',#118199,10.);
#26520=VECTOR('',#118202,1000.);
#26521=VECTOR('',#118205,10.);
#26522=VECTOR('',#118206,1000.);
#26523=VECTOR('',#118209,1000.);
#26524=VECTOR('',#118212,1000.);
#26525=VECTOR('',#118219,10.);
#26526=VECTOR('',#118220,1000.);
#26527=VECTOR('',#118221,10.);
#26528=VECTOR('',#118224,1000.);
#26529=VECTOR('',#118225,10.);
#26530=VECTOR('',#118228,1000.);
#26531=VECTOR('',#118231,10.);
#26532=VECTOR('',#118232,1000.);
#26533=VECTOR('',#118237,10.);
#26534=VECTOR('',#118238,1000.);
#26535=VECTOR('',#118239,10.);
#26536=VECTOR('',#118242,1000.);
#26537=VECTOR('',#118243,10.);
#26538=VECTOR('',#118246,1000.);
#26539=VECTOR('',#118249,10.);
#26540=VECTOR('',#118250,1000.);
#26541=VECTOR('',#118253,1000.);
#26542=VECTOR('',#118256,1000.);
#26543=VECTOR('',#118263,10.);
#26544=VECTOR('',#118264,1000.);
#26545=VECTOR('',#118265,10.);
#26546=VECTOR('',#118268,1000.);
#26547=VECTOR('',#118269,10.);
#26548=VECTOR('',#118272,1000.);
#26549=VECTOR('',#118275,10.);
#26550=VECTOR('',#118276,1000.);
#26551=VECTOR('',#118281,10.);
#26552=VECTOR('',#118282,1000.);
#26553=VECTOR('',#118283,10.);
#26554=VECTOR('',#118286,1000.);
#26555=VECTOR('',#118287,10.);
#26556=VECTOR('',#118290,1000.);
#26557=VECTOR('',#118293,10.);
#26558=VECTOR('',#118294,1000.);
#26559=VECTOR('',#118297,1000.);
#26560=VECTOR('',#118300,1000.);
#26561=VECTOR('',#118307,10.);
#26562=VECTOR('',#118308,1000.);
#26563=VECTOR('',#118309,10.);
#26564=VECTOR('',#118312,1000.);
#26565=VECTOR('',#118313,10.);
#26566=VECTOR('',#118316,1000.);
#26567=VECTOR('',#118319,10.);
#26568=VECTOR('',#118320,1000.);
#26569=VECTOR('',#118325,10.);
#26570=VECTOR('',#118326,1000.);
#26571=VECTOR('',#118327,10.);
#26572=VECTOR('',#118330,1000.);
#26573=VECTOR('',#118331,10.);
#26574=VECTOR('',#118334,1000.);
#26575=VECTOR('',#118337,10.);
#26576=VECTOR('',#118338,1000.);
#26577=VECTOR('',#118341,1000.);
#26578=VECTOR('',#118344,1000.);
#26579=VECTOR('',#118351,10.);
#26580=VECTOR('',#118352,1000.);
#26581=VECTOR('',#118353,10.);
#26582=VECTOR('',#118356,1000.);
#26583=VECTOR('',#118357,10.);
#26584=VECTOR('',#118360,1000.);
#26585=VECTOR('',#118363,10.);
#26586=VECTOR('',#118364,1000.);
#26587=VECTOR('',#118369,10.);
#26588=VECTOR('',#118370,1000.);
#26589=VECTOR('',#118371,10.);
#26590=VECTOR('',#118374,1000.);
#26591=VECTOR('',#118375,10.);
#26592=VECTOR('',#118378,1000.);
#26593=VECTOR('',#118381,10.);
#26594=VECTOR('',#118382,1000.);
#26595=VECTOR('',#118385,1000.);
#26596=VECTOR('',#118388,1000.);
#26597=VECTOR('',#118395,10.);
#26598=VECTOR('',#118396,1000.);
#26599=VECTOR('',#118397,10.);
#26600=VECTOR('',#118400,1000.);
#26601=VECTOR('',#118401,10.);
#26602=VECTOR('',#118404,1000.);
#26603=VECTOR('',#118407,10.);
#26604=VECTOR('',#118408,1000.);
#26605=VECTOR('',#118413,10.);
#26606=VECTOR('',#118414,1000.);
#26607=VECTOR('',#118415,10.);
#26608=VECTOR('',#118418,1000.);
#26609=VECTOR('',#118419,10.);
#26610=VECTOR('',#118422,1000.);
#26611=VECTOR('',#118425,10.);
#26612=VECTOR('',#118426,1000.);
#26613=VECTOR('',#118429,1000.);
#26614=VECTOR('',#118432,1000.);
#26615=VECTOR('',#118439,10.);
#26616=VECTOR('',#118440,1000.);
#26617=VECTOR('',#118441,10.);
#26618=VECTOR('',#118444,1000.);
#26619=VECTOR('',#118445,10.);
#26620=VECTOR('',#118448,1000.);
#26621=VECTOR('',#118451,10.);
#26622=VECTOR('',#118452,1000.);
#26623=VECTOR('',#118457,10.);
#26624=VECTOR('',#118458,1000.);
#26625=VECTOR('',#118459,10.);
#26626=VECTOR('',#118462,1000.);
#26627=VECTOR('',#118463,10.);
#26628=VECTOR('',#118466,1000.);
#26629=VECTOR('',#118469,10.);
#26630=VECTOR('',#118470,1000.);
#26631=VECTOR('',#118473,1000.);
#26632=VECTOR('',#118476,1000.);
#26633=VECTOR('',#118483,10.);
#26634=VECTOR('',#118484,1000.);
#26635=VECTOR('',#118485,10.);
#26636=VECTOR('',#118488,1000.);
#26637=VECTOR('',#118489,10.);
#26638=VECTOR('',#118492,1000.);
#26639=VECTOR('',#118495,10.);
#26640=VECTOR('',#118496,1000.);
#26641=VECTOR('',#118501,10.);
#26642=VECTOR('',#118502,1000.);
#26643=VECTOR('',#118503,10.);
#26644=VECTOR('',#118506,1000.);
#26645=VECTOR('',#118507,10.);
#26646=VECTOR('',#118510,1000.);
#26647=VECTOR('',#118513,10.);
#26648=VECTOR('',#118514,1000.);
#26649=VECTOR('',#118517,1000.);
#26650=VECTOR('',#118520,1000.);
#26651=VECTOR('',#118527,10.);
#26652=VECTOR('',#118528,1000.);
#26653=VECTOR('',#118529,10.);
#26654=VECTOR('',#118532,1000.);
#26655=VECTOR('',#118533,10.);
#26656=VECTOR('',#118536,1000.);
#26657=VECTOR('',#118539,10.);
#26658=VECTOR('',#118540,1000.);
#26659=VECTOR('',#118545,10.);
#26660=VECTOR('',#118546,1000.);
#26661=VECTOR('',#118547,10.);
#26662=VECTOR('',#118550,1000.);
#26663=VECTOR('',#118551,10.);
#26664=VECTOR('',#118554,1000.);
#26665=VECTOR('',#118557,10.);
#26666=VECTOR('',#118558,1000.);
#26667=VECTOR('',#118561,1000.);
#26668=VECTOR('',#118564,1000.);
#26669=VECTOR('',#118571,10.);
#26670=VECTOR('',#118572,1000.);
#26671=VECTOR('',#118573,10.);
#26672=VECTOR('',#118576,1000.);
#26673=VECTOR('',#118577,10.);
#26674=VECTOR('',#118580,1000.);
#26675=VECTOR('',#118583,10.);
#26676=VECTOR('',#118584,1000.);
#26677=VECTOR('',#118589,10.);
#26678=VECTOR('',#118590,1000.);
#26679=VECTOR('',#118591,10.);
#26680=VECTOR('',#118594,1000.);
#26681=VECTOR('',#118595,10.);
#26682=VECTOR('',#118598,1000.);
#26683=VECTOR('',#118601,10.);
#26684=VECTOR('',#118602,1000.);
#26685=VECTOR('',#118605,1000.);
#26686=VECTOR('',#118608,1000.);
#26687=VECTOR('',#118615,10.);
#26688=VECTOR('',#118616,1000.);
#26689=VECTOR('',#118617,10.);
#26690=VECTOR('',#118620,1000.);
#26691=VECTOR('',#118621,10.);
#26692=VECTOR('',#118624,1000.);
#26693=VECTOR('',#118627,10.);
#26694=VECTOR('',#118628,1000.);
#26695=VECTOR('',#118633,10.);
#26696=VECTOR('',#118634,1000.);
#26697=VECTOR('',#118635,10.);
#26698=VECTOR('',#118638,1000.);
#26699=VECTOR('',#118639,10.);
#26700=VECTOR('',#118642,1000.);
#26701=VECTOR('',#118645,10.);
#26702=VECTOR('',#118646,1000.);
#26703=VECTOR('',#118649,1000.);
#26704=VECTOR('',#118652,1000.);
#26705=VECTOR('',#118659,10.);
#26706=VECTOR('',#118660,1000.);
#26707=VECTOR('',#118661,10.);
#26708=VECTOR('',#118664,1000.);
#26709=VECTOR('',#118665,10.);
#26710=VECTOR('',#118668,1000.);
#26711=VECTOR('',#118671,10.);
#26712=VECTOR('',#118672,1000.);
#26713=VECTOR('',#118677,10.);
#26714=VECTOR('',#118678,1000.);
#26715=VECTOR('',#118679,10.);
#26716=VECTOR('',#118682,1000.);
#26717=VECTOR('',#118683,10.);
#26718=VECTOR('',#118686,1000.);
#26719=VECTOR('',#118689,10.);
#26720=VECTOR('',#118690,1000.);
#26721=VECTOR('',#118693,1000.);
#26722=VECTOR('',#118694,1000.);
#26723=VECTOR('',#118699,10.);
#26724=VECTOR('',#118700,1000.);
#26725=VECTOR('',#118701,10.);
#26726=VECTOR('',#118704,1000.);
#26727=VECTOR('',#118705,10.);
#26728=VECTOR('',#118708,1000.);
#26729=VECTOR('',#118711,10.);
#26730=VECTOR('',#118712,1000.);
#26731=VECTOR('',#118717,10.);
#26732=VECTOR('',#118718,1000.);
#26733=VECTOR('',#118719,10.);
#26734=VECTOR('',#118722,1000.);
#26735=VECTOR('',#118723,10.);
#26736=VECTOR('',#118726,1000.);
#26737=VECTOR('',#118729,10.);
#26738=VECTOR('',#118730,1000.);
#26739=VECTOR('',#118733,1000.);
#26740=VECTOR('',#118736,1000.);
#26741=VECTOR('',#118743,10.);
#26742=VECTOR('',#118744,1000.);
#26743=VECTOR('',#118745,10.);
#26744=VECTOR('',#118748,1000.);
#26745=VECTOR('',#118749,10.);
#26746=VECTOR('',#118752,1000.);
#26747=VECTOR('',#118755,10.);
#26748=VECTOR('',#118756,1000.);
#26749=VECTOR('',#118761,10.);
#26750=VECTOR('',#118762,1000.);
#26751=VECTOR('',#118763,10.);
#26752=VECTOR('',#118766,1000.);
#26753=VECTOR('',#118767,10.);
#26754=VECTOR('',#118770,1000.);
#26755=VECTOR('',#118773,10.);
#26756=VECTOR('',#118774,1000.);
#26757=VECTOR('',#118777,1000.);
#26758=VECTOR('',#118780,1000.);
#26759=VECTOR('',#118787,10.);
#26760=VECTOR('',#118788,1000.);
#26761=VECTOR('',#118789,10.);
#26762=VECTOR('',#118792,1000.);
#26763=VECTOR('',#118793,10.);
#26764=VECTOR('',#118796,1000.);
#26765=VECTOR('',#118799,10.);
#26766=VECTOR('',#118800,1000.);
#26767=VECTOR('',#118805,10.);
#26768=VECTOR('',#118806,1000.);
#26769=VECTOR('',#118807,10.);
#26770=VECTOR('',#118810,1000.);
#26771=VECTOR('',#118811,10.);
#26772=VECTOR('',#118814,1000.);
#26773=VECTOR('',#118817,10.);
#26774=VECTOR('',#118818,1000.);
#26775=VECTOR('',#118821,1000.);
#26776=VECTOR('',#118824,1000.);
#26777=VECTOR('',#118831,10.);
#26778=VECTOR('',#118832,1000.);
#26779=VECTOR('',#118833,10.);
#26780=VECTOR('',#118836,1000.);
#26781=VECTOR('',#118837,10.);
#26782=VECTOR('',#118840,1000.);
#26783=VECTOR('',#118843,10.);
#26784=VECTOR('',#118844,1000.);
#26785=VECTOR('',#118849,10.);
#26786=VECTOR('',#118850,1000.);
#26787=VECTOR('',#118851,10.);
#26788=VECTOR('',#118854,1000.);
#26789=VECTOR('',#118855,10.);
#26790=VECTOR('',#118858,1000.);
#26791=VECTOR('',#118861,10.);
#26792=VECTOR('',#118862,1000.);
#26793=VECTOR('',#118865,1000.);
#26794=VECTOR('',#118868,1000.);
#26795=VECTOR('',#118875,10.);
#26796=VECTOR('',#118876,1000.);
#26797=VECTOR('',#118877,10.);
#26798=VECTOR('',#118880,1000.);
#26799=VECTOR('',#118881,10.);
#26800=VECTOR('',#118884,1000.);
#26801=VECTOR('',#118887,10.);
#26802=VECTOR('',#118888,1000.);
#26803=VECTOR('',#118893,10.);
#26804=VECTOR('',#118894,1000.);
#26805=VECTOR('',#118895,10.);
#26806=VECTOR('',#118898,1000.);
#26807=VECTOR('',#118899,10.);
#26808=VECTOR('',#118902,1000.);
#26809=VECTOR('',#118905,10.);
#26810=VECTOR('',#118906,1000.);
#26811=VECTOR('',#118909,1000.);
#26812=VECTOR('',#118912,1000.);
#26813=VECTOR('',#118919,10.);
#26814=VECTOR('',#118920,1000.);
#26815=VECTOR('',#118921,10.);
#26816=VECTOR('',#118924,1000.);
#26817=VECTOR('',#118925,10.);
#26818=VECTOR('',#118928,1000.);
#26819=VECTOR('',#118931,10.);
#26820=VECTOR('',#118932,1000.);
#26821=VECTOR('',#118937,10.);
#26822=VECTOR('',#118938,1000.);
#26823=VECTOR('',#118939,10.);
#26824=VECTOR('',#118942,1000.);
#26825=VECTOR('',#118943,10.);
#26826=VECTOR('',#118946,1000.);
#26827=VECTOR('',#118949,10.);
#26828=VECTOR('',#118950,1000.);
#26829=VECTOR('',#118953,1000.);
#26830=VECTOR('',#118956,1000.);
#26831=VECTOR('',#118963,10.);
#26832=VECTOR('',#118964,1000.);
#26833=VECTOR('',#118965,10.);
#26834=VECTOR('',#118968,1000.);
#26835=VECTOR('',#118969,10.);
#26836=VECTOR('',#118972,1000.);
#26837=VECTOR('',#118975,10.);
#26838=VECTOR('',#118976,1000.);
#26839=VECTOR('',#118981,10.);
#26840=VECTOR('',#118982,1000.);
#26841=VECTOR('',#118983,10.);
#26842=VECTOR('',#118986,1000.);
#26843=VECTOR('',#118987,10.);
#26844=VECTOR('',#118990,1000.);
#26845=VECTOR('',#118993,10.);
#26846=VECTOR('',#118994,1000.);
#26847=VECTOR('',#118997,1000.);
#26848=VECTOR('',#119000,1000.);
#26849=VECTOR('',#119007,10.);
#26850=VECTOR('',#119008,1000.);
#26851=VECTOR('',#119009,10.);
#26852=VECTOR('',#119012,1000.);
#26853=VECTOR('',#119013,10.);
#26854=VECTOR('',#119016,1000.);
#26855=VECTOR('',#119019,10.);
#26856=VECTOR('',#119020,1000.);
#26857=VECTOR('',#119025,10.);
#26858=VECTOR('',#119026,1000.);
#26859=VECTOR('',#119027,10.);
#26860=VECTOR('',#119030,1000.);
#26861=VECTOR('',#119031,10.);
#26862=VECTOR('',#119034,1000.);
#26863=VECTOR('',#119037,10.);
#26864=VECTOR('',#119038,1000.);
#26865=VECTOR('',#119041,1000.);
#26866=VECTOR('',#119044,1000.);
#26867=VECTOR('',#119051,10.);
#26868=VECTOR('',#119052,1000.);
#26869=VECTOR('',#119053,10.);
#26870=VECTOR('',#119056,1000.);
#26871=VECTOR('',#119057,10.);
#26872=VECTOR('',#119060,1000.);
#26873=VECTOR('',#119063,10.);
#26874=VECTOR('',#119064,1000.);
#26875=VECTOR('',#119069,10.);
#26876=VECTOR('',#119070,1000.);
#26877=VECTOR('',#119071,10.);
#26878=VECTOR('',#119074,1000.);
#26879=VECTOR('',#119075,10.);
#26880=VECTOR('',#119078,1000.);
#26881=VECTOR('',#119081,10.);
#26882=VECTOR('',#119082,1000.);
#26883=VECTOR('',#119085,1000.);
#26884=VECTOR('',#119088,1000.);
#26885=VECTOR('',#119095,10.);
#26886=VECTOR('',#119096,1000.);
#26887=VECTOR('',#119097,10.);
#26888=VECTOR('',#119100,1000.);
#26889=VECTOR('',#119101,10.);
#26890=VECTOR('',#119104,1000.);
#26891=VECTOR('',#119107,10.);
#26892=VECTOR('',#119108,1000.);
#26893=VECTOR('',#119113,10.);
#26894=VECTOR('',#119114,1000.);
#26895=VECTOR('',#119115,10.);
#26896=VECTOR('',#119118,1000.);
#26897=VECTOR('',#119119,10.);
#26898=VECTOR('',#119122,1000.);
#26899=VECTOR('',#119125,10.);
#26900=VECTOR('',#119126,1000.);
#26901=VECTOR('',#119129,1000.);
#26902=VECTOR('',#119132,1000.);
#26903=VECTOR('',#119139,10.);
#26904=VECTOR('',#119140,1000.);
#26905=VECTOR('',#119141,10.);
#26906=VECTOR('',#119144,1000.);
#26907=VECTOR('',#119145,10.);
#26908=VECTOR('',#119148,1000.);
#26909=VECTOR('',#119151,10.);
#26910=VECTOR('',#119152,1000.);
#26911=VECTOR('',#119157,10.);
#26912=VECTOR('',#119158,1000.);
#26913=VECTOR('',#119159,10.);
#26914=VECTOR('',#119162,1000.);
#26915=VECTOR('',#119163,10.);
#26916=VECTOR('',#119166,1000.);
#26917=VECTOR('',#119169,10.);
#26918=VECTOR('',#119170,1000.);
#26919=VECTOR('',#119173,1000.);
#26920=VECTOR('',#119176,1000.);
#26921=VECTOR('',#119183,10.);
#26922=VECTOR('',#119184,1000.);
#26923=VECTOR('',#119185,10.);
#26924=VECTOR('',#119188,1000.);
#26925=VECTOR('',#119189,10.);
#26926=VECTOR('',#119192,1000.);
#26927=VECTOR('',#119195,10.);
#26928=VECTOR('',#119196,1000.);
#26929=VECTOR('',#119201,10.);
#26930=VECTOR('',#119202,1000.);
#26931=VECTOR('',#119203,10.);
#26932=VECTOR('',#119206,1000.);
#26933=VECTOR('',#119207,10.);
#26934=VECTOR('',#119210,1000.);
#26935=VECTOR('',#119213,10.);
#26936=VECTOR('',#119214,1000.);
#26937=VECTOR('',#119217,1000.);
#26938=VECTOR('',#119220,1000.);
#26939=VECTOR('',#119227,10.);
#26940=VECTOR('',#119228,1000.);
#26941=VECTOR('',#119229,10.);
#26942=VECTOR('',#119232,1000.);
#26943=VECTOR('',#119233,10.);
#26944=VECTOR('',#119236,1000.);
#26945=VECTOR('',#119239,10.);
#26946=VECTOR('',#119240,1000.);
#26947=VECTOR('',#119245,10.);
#26948=VECTOR('',#119246,1000.);
#26949=VECTOR('',#119247,10.);
#26950=VECTOR('',#119250,1000.);
#26951=VECTOR('',#119251,10.);
#26952=VECTOR('',#119254,1000.);
#26953=VECTOR('',#119257,10.);
#26954=VECTOR('',#119258,1000.);
#26955=VECTOR('',#119261,1000.);
#26956=VECTOR('',#119264,1000.);
#26957=VECTOR('',#119271,10.);
#26958=VECTOR('',#119272,1000.);
#26959=VECTOR('',#119273,10.);
#26960=VECTOR('',#119276,1000.);
#26961=VECTOR('',#119277,10.);
#26962=VECTOR('',#119280,1000.);
#26963=VECTOR('',#119283,10.);
#26964=VECTOR('',#119284,1000.);
#26965=VECTOR('',#119289,10.);
#26966=VECTOR('',#119290,1000.);
#26967=VECTOR('',#119291,10.);
#26968=VECTOR('',#119294,1000.);
#26969=VECTOR('',#119295,10.);
#26970=VECTOR('',#119298,1000.);
#26971=VECTOR('',#119301,10.);
#26972=VECTOR('',#119302,1000.);
#26973=VECTOR('',#119305,1000.);
#26974=VECTOR('',#119308,1000.);
#26975=VECTOR('',#119315,10.);
#26976=VECTOR('',#119316,1000.);
#26977=VECTOR('',#119317,10.);
#26978=VECTOR('',#119320,1000.);
#26979=VECTOR('',#119321,10.);
#26980=VECTOR('',#119324,1000.);
#26981=VECTOR('',#119327,10.);
#26982=VECTOR('',#119328,1000.);
#26983=VECTOR('',#119333,10.);
#26984=VECTOR('',#119334,1000.);
#26985=VECTOR('',#119335,10.);
#26986=VECTOR('',#119338,1000.);
#26987=VECTOR('',#119339,10.);
#26988=VECTOR('',#119342,1000.);
#26989=VECTOR('',#119345,10.);
#26990=VECTOR('',#119346,1000.);
#26991=VECTOR('',#119349,1000.);
#26992=VECTOR('',#119350,1000.);
#26993=VECTOR('',#119355,10.);
#26994=VECTOR('',#119356,1000.);
#26995=VECTOR('',#119357,10.);
#26996=VECTOR('',#119360,1000.);
#26997=VECTOR('',#119361,10.);
#26998=VECTOR('',#119364,1000.);
#26999=VECTOR('',#119367,10.);
#27000=VECTOR('',#119368,1000.);
#27001=VECTOR('',#119373,10.);
#27002=VECTOR('',#119374,1000.);
#27003=VECTOR('',#119375,10.);
#27004=VECTOR('',#119378,1000.);
#27005=VECTOR('',#119379,10.);
#27006=VECTOR('',#119382,1000.);
#27007=VECTOR('',#119385,10.);
#27008=VECTOR('',#119386,1000.);
#27009=VECTOR('',#119389,1000.);
#27010=VECTOR('',#119392,1000.);
#27011=VECTOR('',#119399,10.);
#27012=VECTOR('',#119400,1000.);
#27013=VECTOR('',#119401,10.);
#27014=VECTOR('',#119404,1000.);
#27015=VECTOR('',#119405,10.);
#27016=VECTOR('',#119408,1000.);
#27017=VECTOR('',#119411,10.);
#27018=VECTOR('',#119412,1000.);
#27019=VECTOR('',#119417,10.);
#27020=VECTOR('',#119418,1000.);
#27021=VECTOR('',#119419,10.);
#27022=VECTOR('',#119422,1000.);
#27023=VECTOR('',#119423,10.);
#27024=VECTOR('',#119426,1000.);
#27025=VECTOR('',#119429,10.);
#27026=VECTOR('',#119430,1000.);
#27027=VECTOR('',#119433,1000.);
#27028=VECTOR('',#119436,1000.);
#27029=VECTOR('',#119443,10.);
#27030=VECTOR('',#119444,1000.);
#27031=VECTOR('',#119445,10.);
#27032=VECTOR('',#119448,1000.);
#27033=VECTOR('',#119449,10.);
#27034=VECTOR('',#119452,1000.);
#27035=VECTOR('',#119455,10.);
#27036=VECTOR('',#119456,1000.);
#27037=VECTOR('',#119461,10.);
#27038=VECTOR('',#119462,1000.);
#27039=VECTOR('',#119463,10.);
#27040=VECTOR('',#119466,1000.);
#27041=VECTOR('',#119467,10.);
#27042=VECTOR('',#119470,1000.);
#27043=VECTOR('',#119473,10.);
#27044=VECTOR('',#119474,1000.);
#27045=VECTOR('',#119477,1000.);
#27046=VECTOR('',#119480,1000.);
#27047=VECTOR('',#119487,10.);
#27048=VECTOR('',#119488,1000.);
#27049=VECTOR('',#119489,10.);
#27050=VECTOR('',#119492,1000.);
#27051=VECTOR('',#119493,10.);
#27052=VECTOR('',#119496,1000.);
#27053=VECTOR('',#119499,10.);
#27054=VECTOR('',#119500,1000.);
#27055=VECTOR('',#119505,10.);
#27056=VECTOR('',#119506,1000.);
#27057=VECTOR('',#119507,10.);
#27058=VECTOR('',#119510,1000.);
#27059=VECTOR('',#119511,10.);
#27060=VECTOR('',#119514,1000.);
#27061=VECTOR('',#119517,10.);
#27062=VECTOR('',#119518,1000.);
#27063=VECTOR('',#119521,1000.);
#27064=VECTOR('',#119524,1000.);
#27065=VECTOR('',#119531,10.);
#27066=VECTOR('',#119532,1000.);
#27067=VECTOR('',#119533,10.);
#27068=VECTOR('',#119536,1000.);
#27069=VECTOR('',#119537,10.);
#27070=VECTOR('',#119540,1000.);
#27071=VECTOR('',#119543,10.);
#27072=VECTOR('',#119544,1000.);
#27073=VECTOR('',#119549,10.);
#27074=VECTOR('',#119550,1000.);
#27075=VECTOR('',#119551,10.);
#27076=VECTOR('',#119554,1000.);
#27077=VECTOR('',#119555,10.);
#27078=VECTOR('',#119558,1000.);
#27079=VECTOR('',#119561,10.);
#27080=VECTOR('',#119562,1000.);
#27081=VECTOR('',#119565,1000.);
#27082=VECTOR('',#119568,1000.);
#27083=VECTOR('',#119575,10.);
#27084=VECTOR('',#119576,1000.);
#27085=VECTOR('',#119577,10.);
#27086=VECTOR('',#119580,1000.);
#27087=VECTOR('',#119581,10.);
#27088=VECTOR('',#119584,1000.);
#27089=VECTOR('',#119587,10.);
#27090=VECTOR('',#119588,1000.);
#27091=VECTOR('',#119593,10.);
#27092=VECTOR('',#119594,1000.);
#27093=VECTOR('',#119595,10.);
#27094=VECTOR('',#119598,1000.);
#27095=VECTOR('',#119599,10.);
#27096=VECTOR('',#119602,1000.);
#27097=VECTOR('',#119605,10.);
#27098=VECTOR('',#119606,1000.);
#27099=VECTOR('',#119609,1000.);
#27100=VECTOR('',#119612,1000.);
#27101=VECTOR('',#119619,10.);
#27102=VECTOR('',#119620,1000.);
#27103=VECTOR('',#119621,10.);
#27104=VECTOR('',#119624,1000.);
#27105=VECTOR('',#119625,10.);
#27106=VECTOR('',#119628,1000.);
#27107=VECTOR('',#119631,10.);
#27108=VECTOR('',#119632,1000.);
#27109=VECTOR('',#119637,10.);
#27110=VECTOR('',#119638,1000.);
#27111=VECTOR('',#119639,10.);
#27112=VECTOR('',#119642,1000.);
#27113=VECTOR('',#119643,10.);
#27114=VECTOR('',#119646,1000.);
#27115=VECTOR('',#119649,10.);
#27116=VECTOR('',#119650,1000.);
#27117=VECTOR('',#119653,1000.);
#27118=VECTOR('',#119656,1000.);
#27119=VECTOR('',#119663,10.);
#27120=VECTOR('',#119664,1000.);
#27121=VECTOR('',#119665,10.);
#27122=VECTOR('',#119668,1000.);
#27123=VECTOR('',#119669,10.);
#27124=VECTOR('',#119672,1000.);
#27125=VECTOR('',#119675,10.);
#27126=VECTOR('',#119676,1000.);
#27127=VECTOR('',#119681,10.);
#27128=VECTOR('',#119682,1000.);
#27129=VECTOR('',#119683,10.);
#27130=VECTOR('',#119686,1000.);
#27131=VECTOR('',#119687,10.);
#27132=VECTOR('',#119690,1000.);
#27133=VECTOR('',#119693,10.);
#27134=VECTOR('',#119694,1000.);
#27135=VECTOR('',#119697,1000.);
#27136=VECTOR('',#119700,1000.);
#27137=VECTOR('',#119707,10.);
#27138=VECTOR('',#119708,1000.);
#27139=VECTOR('',#119709,10.);
#27140=VECTOR('',#119712,1000.);
#27141=VECTOR('',#119713,10.);
#27142=VECTOR('',#119716,1000.);
#27143=VECTOR('',#119719,10.);
#27144=VECTOR('',#119720,1000.);
#27145=VECTOR('',#119725,10.);
#27146=VECTOR('',#119726,1000.);
#27147=VECTOR('',#119727,10.);
#27148=VECTOR('',#119730,1000.);
#27149=VECTOR('',#119731,10.);
#27150=VECTOR('',#119734,1000.);
#27151=VECTOR('',#119737,10.);
#27152=VECTOR('',#119738,1000.);
#27153=VECTOR('',#119741,1000.);
#27154=VECTOR('',#119744,1000.);
#27155=VECTOR('',#119751,10.);
#27156=VECTOR('',#119752,1000.);
#27157=VECTOR('',#119753,10.);
#27158=VECTOR('',#119756,1000.);
#27159=VECTOR('',#119757,10.);
#27160=VECTOR('',#119760,1000.);
#27161=VECTOR('',#119763,10.);
#27162=VECTOR('',#119764,1000.);
#27163=VECTOR('',#119769,10.);
#27164=VECTOR('',#119770,1000.);
#27165=VECTOR('',#119771,10.);
#27166=VECTOR('',#119774,1000.);
#27167=VECTOR('',#119775,10.);
#27168=VECTOR('',#119778,1000.);
#27169=VECTOR('',#119781,10.);
#27170=VECTOR('',#119782,1000.);
#27171=VECTOR('',#119785,1000.);
#27172=VECTOR('',#119788,1000.);
#27173=VECTOR('',#119795,10.);
#27174=VECTOR('',#119796,1000.);
#27175=VECTOR('',#119797,10.);
#27176=VECTOR('',#119800,1000.);
#27177=VECTOR('',#119801,10.);
#27178=VECTOR('',#119804,1000.);
#27179=VECTOR('',#119807,10.);
#27180=VECTOR('',#119808,1000.);
#27181=VECTOR('',#119813,10.);
#27182=VECTOR('',#119814,1000.);
#27183=VECTOR('',#119815,10.);
#27184=VECTOR('',#119818,1000.);
#27185=VECTOR('',#119819,10.);
#27186=VECTOR('',#119822,1000.);
#27187=VECTOR('',#119825,10.);
#27188=VECTOR('',#119826,1000.);
#27189=VECTOR('',#119829,1000.);
#27190=VECTOR('',#119832,1000.);
#27191=VECTOR('',#119839,10.);
#27192=VECTOR('',#119840,1000.);
#27193=VECTOR('',#119841,10.);
#27194=VECTOR('',#119844,1000.);
#27195=VECTOR('',#119845,10.);
#27196=VECTOR('',#119848,1000.);
#27197=VECTOR('',#119851,10.);
#27198=VECTOR('',#119852,1000.);
#27199=VECTOR('',#119857,10.);
#27200=VECTOR('',#119858,1000.);
#27201=VECTOR('',#119859,10.);
#27202=VECTOR('',#119862,1000.);
#27203=VECTOR('',#119863,10.);
#27204=VECTOR('',#119866,1000.);
#27205=VECTOR('',#119869,10.);
#27206=VECTOR('',#119870,1000.);
#27207=VECTOR('',#119873,1000.);
#27208=VECTOR('',#119876,1000.);
#27209=VECTOR('',#119883,10.);
#27210=VECTOR('',#119884,1000.);
#27211=VECTOR('',#119885,10.);
#27212=VECTOR('',#119888,1000.);
#27213=VECTOR('',#119889,10.);
#27214=VECTOR('',#119892,1000.);
#27215=VECTOR('',#119895,10.);
#27216=VECTOR('',#119896,1000.);
#27217=VECTOR('',#119901,10.);
#27218=VECTOR('',#119902,1000.);
#27219=VECTOR('',#119903,10.);
#27220=VECTOR('',#119906,1000.);
#27221=VECTOR('',#119907,10.);
#27222=VECTOR('',#119910,1000.);
#27223=VECTOR('',#119913,10.);
#27224=VECTOR('',#119914,1000.);
#27225=VECTOR('',#119917,1000.);
#27226=VECTOR('',#119920,1000.);
#27227=VECTOR('',#119927,10.);
#27228=VECTOR('',#119928,1000.);
#27229=VECTOR('',#119929,10.);
#27230=VECTOR('',#119932,1000.);
#27231=VECTOR('',#119933,10.);
#27232=VECTOR('',#119936,1000.);
#27233=VECTOR('',#119939,10.);
#27234=VECTOR('',#119940,1000.);
#27235=VECTOR('',#119945,10.);
#27236=VECTOR('',#119946,1000.);
#27237=VECTOR('',#119947,10.);
#27238=VECTOR('',#119950,1000.);
#27239=VECTOR('',#119951,10.);
#27240=VECTOR('',#119954,1000.);
#27241=VECTOR('',#119957,10.);
#27242=VECTOR('',#119958,1000.);
#27243=VECTOR('',#119961,1000.);
#27244=VECTOR('',#119964,1000.);
#27245=VECTOR('',#119971,10.);
#27246=VECTOR('',#119972,1000.);
#27247=VECTOR('',#119973,10.);
#27248=VECTOR('',#119976,1000.);
#27249=VECTOR('',#119977,10.);
#27250=VECTOR('',#119980,1000.);
#27251=VECTOR('',#119983,10.);
#27252=VECTOR('',#119984,1000.);
#27253=VECTOR('',#119989,10.);
#27254=VECTOR('',#119990,1000.);
#27255=VECTOR('',#119991,10.);
#27256=VECTOR('',#119994,1000.);
#27257=VECTOR('',#119995,10.);
#27258=VECTOR('',#119998,1000.);
#27259=VECTOR('',#120001,10.);
#27260=VECTOR('',#120002,1000.);
#27261=VECTOR('',#125489,65.);
#27262=VECTOR('',#125494,64.008019903844);
#27263=VECTOR('',#125499,10.);
#27264=VECTOR('',#125502,10.);
#27265=VECTOR('',#125505,10.);
#27266=VECTOR('',#125508,10.);
#27267=VECTOR('',#125511,10.);
#27268=VECTOR('',#125514,10.);
#27269=VECTOR('',#125517,10.);
#27270=VECTOR('',#125520,10.);
#27271=VECTOR('',#125523,10.);
#27272=VECTOR('',#125526,10.);
#27273=VECTOR('',#125529,10.);
#27274=VECTOR('',#125532,10.);
#27275=VECTOR('',#125535,10.);
#27276=VECTOR('',#125538,10.);
#27277=VECTOR('',#125541,10.);
#27278=VECTOR('',#125544,10.);
#27279=VECTOR('',#125547,10.);
#27280=VECTOR('',#125550,10.);
#27281=VECTOR('',#125553,10.);
#27282=VECTOR('',#125556,10.);
#27283=VECTOR('',#125559,10.);
#27284=VECTOR('',#125562,10.);
#27285=VECTOR('',#125565,10.);
#27286=VECTOR('',#125568,10.);
#27287=VECTOR('',#125571,10.);
#27288=VECTOR('',#125574,10.);
#27289=VECTOR('',#125577,10.);
#27290=VECTOR('',#125580,10.);
#27291=VECTOR('',#125583,10.);
#27292=VECTOR('',#125586,10.);
#27293=VECTOR('',#125589,10.);
#27294=VECTOR('',#125592,10.);
#27295=VECTOR('',#125595,10.);
#27296=VECTOR('',#125598,10.);
#27297=VECTOR('',#125601,10.);
#27298=VECTOR('',#125604,10.);
#27299=VECTOR('',#125607,10.);
#27300=VECTOR('',#125610,10.);
#27301=VECTOR('',#125613,10.);
#27302=VECTOR('',#125616,10.);
#27303=VECTOR('',#125619,10.);
#27304=VECTOR('',#125622,10.);
#27305=VECTOR('',#125625,10.);
#27306=VECTOR('',#125628,10.);
#27307=VECTOR('',#125631,10.);
#27308=VECTOR('',#125634,10.);
#27309=VECTOR('',#125637,10.);
#27310=VECTOR('',#125640,10.);
#27311=VECTOR('',#125643,10.);
#27312=VECTOR('',#125646,10.);
#27313=VECTOR('',#125649,10.);
#27314=VECTOR('',#125652,10.);
#27315=VECTOR('',#125655,10.);
#27316=VECTOR('',#125658,10.);
#27317=VECTOR('',#125661,10.);
#27318=VECTOR('',#125664,10.);
#27319=VECTOR('',#125667,10.);
#27320=VECTOR('',#125670,10.);
#27321=VECTOR('',#125673,10.);
#27322=VECTOR('',#125676,10.);
#27323=VECTOR('',#125677,62.2224557307631);
#27324=VECTOR('',#125678,10.);
#27325=VECTOR('',#125681,10.);
#27326=VECTOR('',#125684,10.);
#27327=VECTOR('',#125687,10.);
#27328=VECTOR('',#125690,10.);
#27329=VECTOR('',#125693,10.);
#27330=VECTOR('',#125696,10.);
#27331=VECTOR('',#125699,10.);
#27332=VECTOR('',#125702,10.);
#27333=VECTOR('',#125705,10.);
#27334=VECTOR('',#125708,10.);
#27335=VECTOR('',#125711,10.);
#27336=VECTOR('',#125714,10.);
#27337=VECTOR('',#125717,10.);
#27338=VECTOR('',#125720,10.);
#27339=VECTOR('',#125723,10.);
#27340=VECTOR('',#125726,10.);
#27341=VECTOR('',#125729,10.);
#27342=VECTOR('',#125732,10.);
#27343=VECTOR('',#125735,10.);
#27344=VECTOR('',#125738,10.);
#27345=VECTOR('',#125741,10.);
#27346=VECTOR('',#125744,10.);
#27347=VECTOR('',#125747,10.);
#27348=VECTOR('',#125750,10.);
#27349=VECTOR('',#125753,10.);
#27350=VECTOR('',#125756,10.);
#27351=VECTOR('',#125759,10.);
#27352=VECTOR('',#125762,10.);
#27353=VECTOR('',#125765,10.);
#27354=VECTOR('',#125766,10.);
#27355=VECTOR('',#125769,10.);
#27356=VECTOR('',#125772,10.);
#27357=VECTOR('',#125775,10.);
#27358=VECTOR('',#125778,10.);
#27359=VECTOR('',#125781,10.);
#27360=VECTOR('',#125784,10.);
#27361=VECTOR('',#125787,10.);
#27362=VECTOR('',#125790,10.);
#27363=VECTOR('',#125793,10.);
#27364=VECTOR('',#125796,10.);
#27365=VECTOR('',#125799,10.);
#27366=VECTOR('',#125802,10.);
#27367=VECTOR('',#125805,10.);
#27368=VECTOR('',#125808,10.);
#27369=VECTOR('',#125811,10.);
#27370=VECTOR('',#125814,10.);
#27371=VECTOR('',#125817,10.);
#27372=VECTOR('',#125820,10.);
#27373=VECTOR('',#125823,10.);
#27374=VECTOR('',#125826,10.);
#27375=VECTOR('',#125829,10.);
#27376=VECTOR('',#125832,10.);
#27377=VECTOR('',#125835,10.);
#27378=VECTOR('',#125838,10.);
#27379=VECTOR('',#125841,10.);
#27380=VECTOR('',#125844,10.);
#27381=VECTOR('',#125847,10.);
#27382=VECTOR('',#125850,10.);
#27383=VECTOR('',#125853,10.);
#27384=VECTOR('',#125856,10.);
#27385=VECTOR('',#125859,10.);
#27386=VECTOR('',#125862,10.);
#27387=VECTOR('',#125865,10.);
#27388=VECTOR('',#125868,10.);
#27389=VECTOR('',#125871,10.);
#27390=VECTOR('',#125874,10.);
#27391=VECTOR('',#125877,10.);
#27392=VECTOR('',#125880,10.);
#27393=VECTOR('',#125883,10.);
#27394=VECTOR('',#125886,10.);
#27395=VECTOR('',#125889,10.);
#27396=VECTOR('',#125892,10.);
#27397=VECTOR('',#125895,10.);
#27398=VECTOR('',#125898,10.);
#27399=VECTOR('',#125901,10.);
#27400=VECTOR('',#125904,10.);
#27401=VECTOR('',#125907,10.);
#27402=VECTOR('',#125910,10.);
#27403=VECTOR('',#125913,10.);
#27404=VECTOR('',#125916,10.);
#27405=VECTOR('',#125919,10.);
#27406=VECTOR('',#125922,10.);
#27407=VECTOR('',#125925,10.);
#27408=VECTOR('',#125928,10.);
#27409=VECTOR('',#125931,10.);
#27410=VECTOR('',#125934,10.);
#27411=VECTOR('',#125937,10.);
#27412=VECTOR('',#125940,10.);
#27413=VECTOR('',#125943,10.);
#27414=VECTOR('',#125946,10.);
#27415=VECTOR('',#125949,10.);
#27416=VECTOR('',#125952,10.);
#27417=VECTOR('',#125955,10.);
#27418=VECTOR('',#125958,10.);
#27419=VECTOR('',#125961,10.);
#27420=VECTOR('',#125964,10.);
#27421=VECTOR('',#125967,10.);
#27422=VECTOR('',#125970,10.);
#27423=VECTOR('',#125973,10.);
#27424=VECTOR('',#125976,10.);
#27425=VECTOR('',#125979,10.);
#27426=VECTOR('',#125982,10.);
#27427=VECTOR('',#125985,10.);
#27428=VECTOR('',#125988,10.);
#27429=VECTOR('',#125991,10.);
#27430=VECTOR('',#125994,10.);
#27431=VECTOR('',#125997,10.);
#27432=VECTOR('',#126000,10.);
#27433=VECTOR('',#126003,10.);
#27434=VECTOR('',#126006,10.);
#27435=VECTOR('',#126009,10.);
#27436=VECTOR('',#126012,10.);
#27437=VECTOR('',#126015,10.);
#27438=VECTOR('',#126018,10.);
#27439=VECTOR('',#126021,10.);
#27440=VECTOR('',#126024,10.);
#27441=VECTOR('',#126027,10.);
#27442=VECTOR('',#126030,10.);
#27443=VECTOR('',#126033,10.);
#27444=VECTOR('',#126036,58.6605641730809);
#27445=VECTOR('',#126039,10.);
#27446=VECTOR('',#126042,10.);
#27447=VECTOR('',#126045,10.);
#27448=VECTOR('',#126048,10.);
#27449=VECTOR('',#126051,10.);
#27450=VECTOR('',#126054,10.);
#27451=VECTOR('',#126057,10.);
#27452=VECTOR('',#126060,10.);
#27453=VECTOR('',#126063,10.);
#27454=VECTOR('',#126066,10.);
#27455=VECTOR('',#126069,10.);
#27456=VECTOR('',#126072,10.);
#27457=VECTOR('',#126075,10.);
#27458=VECTOR('',#126078,10.);
#27459=VECTOR('',#126081,10.);
#27460=VECTOR('',#126084,10.);
#27461=VECTOR('',#126087,10.);
#27462=VECTOR('',#126090,10.);
#27463=VECTOR('',#126093,10.);
#27464=VECTOR('',#126096,10.);
#27465=VECTOR('',#126099,10.);
#27466=VECTOR('',#126102,10.);
#27467=VECTOR('',#126105,10.);
#27468=VECTOR('',#126108,10.);
#27469=VECTOR('',#126111,10.);
#27470=VECTOR('',#126114,10.);
#27471=VECTOR('',#126117,10.);
#27472=VECTOR('',#126120,10.);
#27473=VECTOR('',#126123,10.);
#27474=VECTOR('',#126126,10.);
#27475=VECTOR('',#126127,10.);
#27476=VECTOR('',#126130,10.);
#27477=VECTOR('',#126133,10.);
#27478=VECTOR('',#126136,10.);
#27479=VECTOR('',#126139,10.);
#27480=VECTOR('',#126142,10.);
#27481=VECTOR('',#126145,10.);
#27482=VECTOR('',#126148,10.);
#27483=VECTOR('',#126151,10.);
#27484=VECTOR('',#126154,10.);
#27485=VECTOR('',#126157,10.);
#27486=VECTOR('',#126160,10.);
#27487=VECTOR('',#126163,10.);
#27488=VECTOR('',#126166,10.);
#27489=VECTOR('',#126169,10.);
#27490=VECTOR('',#126172,10.);
#27491=VECTOR('',#126175,10.);
#27492=VECTOR('',#126178,10.);
#27493=VECTOR('',#126181,10.);
#27494=VECTOR('',#126184,10.);
#27495=VECTOR('',#126187,10.);
#27496=VECTOR('',#126190,10.);
#27497=VECTOR('',#126193,10.);
#27498=VECTOR('',#126196,10.);
#27499=VECTOR('',#126199,10.);
#27500=VECTOR('',#126202,10.);
#27501=VECTOR('',#126205,10.);
#27502=VECTOR('',#126208,10.);
#27503=VECTOR('',#126211,10.);
#27504=VECTOR('',#126214,10.);
#27505=VECTOR('',#126219,56.875);
#27506=VECTOR('',#126224,56.875);
#27507=VECTOR('',#126231,1000.);
#27508=VECTOR('',#126234,1000.);
#27509=VECTOR('',#126243,10.);
#27510=VECTOR('',#126244,10.);
#27511=VECTOR('',#126249,1000.);
#27512=VECTOR('',#126252,1000.);
#27513=VECTOR('',#126257,10.);
#27514=VECTOR('',#126260,10.);
#27515=VECTOR('',#126269,1000.);
#27516=VECTOR('',#126270,1000.);
#27517=VECTOR('',#126299,1000.);
#27518=VECTOR('',#126306,1000.);
#27519=VECTOR('',#126309,10.);
#27520=VECTOR('',#126312,10.);
#27521=VECTOR('',#126317,1000.);
#27522=VECTOR('',#126320,1000.);
#27523=VECTOR('',#126325,10.);
#27524=VECTOR('',#126332,10.);
#27525=VECTOR('',#126335,1000.);
#27526=VECTOR('',#126338,1000.);
#27527=VECTOR('',#126367,1000.);
#27528=VECTOR('',#126374,1000.);
#27529=VECTOR('',#126377,10.);
#27530=VECTOR('',#126380,10.);
#27531=VECTOR('',#126385,1000.);
#27532=VECTOR('',#126388,1000.);
#27533=VECTOR('',#126393,10.);
#27534=VECTOR('',#126400,10.);
#27535=VECTOR('',#126403,1000.);
#27536=VECTOR('',#126406,1000.);
#27537=VECTOR('',#126435,1000.);
#27538=VECTOR('',#126442,1000.);
#27539=VECTOR('',#126445,10.);
#27540=VECTOR('',#126448,10.);
#27541=VECTOR('',#126453,1000.);
#27542=VECTOR('',#126456,1000.);
#27543=VECTOR('',#126461,10.);
#27544=VECTOR('',#126468,10.);
#27545=VECTOR('',#126471,1000.);
#27546=VECTOR('',#126474,1000.);
#27547=VECTOR('',#126503,1000.);
#27548=VECTOR('',#126510,1000.);
#27549=VECTOR('',#126513,10.);
#27550=VECTOR('',#126516,10.);
#27551=VECTOR('',#126521,1000.);
#27552=VECTOR('',#126524,1000.);
#27553=VECTOR('',#126529,10.);
#27554=VECTOR('',#126536,10.);
#27555=VECTOR('',#126539,1000.);
#27556=VECTOR('',#126542,1000.);
#27557=VECTOR('',#126571,1000.);
#27558=VECTOR('',#126578,1000.);
#27559=VECTOR('',#126581,10.);
#27560=VECTOR('',#126584,10.);
#27561=VECTOR('',#126589,1000.);
#27562=VECTOR('',#126592,1000.);
#27563=VECTOR('',#126597,10.);
#27564=VECTOR('',#126604,10.);
#27565=VECTOR('',#126607,1000.);
#27566=VECTOR('',#126610,1000.);
#27567=VECTOR('',#126639,1000.);
#27568=VECTOR('',#126646,1000.);
#27569=VECTOR('',#126649,10.);
#27570=VECTOR('',#126652,10.);
#27571=VECTOR('',#126657,1000.);
#27572=VECTOR('',#126660,1000.);
#27573=VECTOR('',#126665,10.);
#27574=VECTOR('',#126672,10.);
#27575=VECTOR('',#126675,1000.);
#27576=VECTOR('',#126678,1000.);
#27577=VECTOR('',#126707,1000.);
#27578=VECTOR('',#126714,1000.);
#27579=VECTOR('',#126717,10.);
#27580=VECTOR('',#126720,10.);
#27581=VECTOR('',#126725,1000.);
#27582=VECTOR('',#126728,1000.);
#27583=VECTOR('',#126733,10.);
#27584=VECTOR('',#126740,10.);
#27585=VECTOR('',#126743,1000.);
#27586=VECTOR('',#126746,1000.);
#27587=VECTOR('',#126775,1000.);
#27588=VECTOR('',#126782,1000.);
#27589=VECTOR('',#126785,10.);
#27590=VECTOR('',#126788,10.);
#27591=VECTOR('',#126793,1000.);
#27592=VECTOR('',#126796,1000.);
#27593=VECTOR('',#126801,10.);
#27594=VECTOR('',#126808,10.);
#27595=VECTOR('',#126811,1000.);
#27596=VECTOR('',#126814,1000.);
#27597=VECTOR('',#126843,1000.);
#27598=VECTOR('',#126850,1000.);
#27599=VECTOR('',#126853,10.);
#27600=VECTOR('',#126856,10.);
#27601=VECTOR('',#126861,1000.);
#27602=VECTOR('',#126864,1000.);
#27603=VECTOR('',#126869,10.);
#27604=VECTOR('',#126876,10.);
#27605=VECTOR('',#126879,1000.);
#27606=VECTOR('',#126882,1000.);
#27607=VECTOR('',#126911,1000.);
#27608=VECTOR('',#126918,1000.);
#27609=VECTOR('',#126921,10.);
#27610=VECTOR('',#126924,10.);
#27611=VECTOR('',#126929,1000.);
#27612=VECTOR('',#126932,1000.);
#27613=VECTOR('',#126937,10.);
#27614=VECTOR('',#126944,10.);
#27615=VECTOR('',#126947,1000.);
#27616=VECTOR('',#126950,1000.);
#27617=VECTOR('',#126979,1000.);
#27618=VECTOR('',#126986,1000.);
#27619=VECTOR('',#126989,10.);
#27620=VECTOR('',#126992,10.);
#27621=VECTOR('',#126997,1000.);
#27622=VECTOR('',#127000,1000.);
#27623=VECTOR('',#127005,10.);
#27624=VECTOR('',#127012,10.);
#27625=VECTOR('',#127015,1000.);
#27626=VECTOR('',#127018,1000.);
#27627=VECTOR('',#127047,1000.);
#27628=VECTOR('',#127054,1000.);
#27629=VECTOR('',#127057,10.);
#27630=VECTOR('',#127060,10.);
#27631=VECTOR('',#127065,1000.);
#27632=VECTOR('',#127068,1000.);
#27633=VECTOR('',#127073,10.);
#27634=VECTOR('',#127080,10.);
#27635=VECTOR('',#127083,1000.);
#27636=VECTOR('',#127086,1000.);
#27637=VECTOR('',#127115,1000.);
#27638=VECTOR('',#127122,1000.);
#27639=VECTOR('',#127125,10.);
#27640=VECTOR('',#127128,10.);
#27641=VECTOR('',#127133,1000.);
#27642=VECTOR('',#127136,1000.);
#27643=VECTOR('',#127141,10.);
#27644=VECTOR('',#127148,10.);
#27645=VECTOR('',#127151,1000.);
#27646=VECTOR('',#127154,1000.);
#27647=VECTOR('',#127183,1000.);
#27648=VECTOR('',#127190,1000.);
#27649=VECTOR('',#127193,10.);
#27650=VECTOR('',#127196,10.);
#27651=VECTOR('',#127201,1000.);
#27652=VECTOR('',#127204,1000.);
#27653=VECTOR('',#127209,10.);
#27654=VECTOR('',#127216,10.);
#27655=VECTOR('',#127219,1000.);
#27656=VECTOR('',#127222,1000.);
#27657=VECTOR('',#127251,1000.);
#27658=VECTOR('',#127258,1000.);
#27659=VECTOR('',#127261,10.);
#27660=VECTOR('',#127264,10.);
#27661=VECTOR('',#127269,1000.);
#27662=VECTOR('',#127272,1000.);
#27663=VECTOR('',#127277,10.);
#27664=VECTOR('',#127284,10.);
#27665=VECTOR('',#127287,1000.);
#27666=VECTOR('',#127290,1000.);
#27667=VECTOR('',#127319,1000.);
#27668=VECTOR('',#127326,1000.);
#27669=VECTOR('',#127329,10.);
#27670=VECTOR('',#127332,10.);
#27671=VECTOR('',#127337,1000.);
#27672=VECTOR('',#127340,1000.);
#27673=VECTOR('',#127345,10.);
#27674=VECTOR('',#127352,10.);
#27675=VECTOR('',#127355,1000.);
#27676=VECTOR('',#127358,1000.);
#27677=VECTOR('',#127387,1000.);
#27678=VECTOR('',#127394,1000.);
#27679=VECTOR('',#127397,10.);
#27680=VECTOR('',#127400,10.);
#27681=VECTOR('',#127405,1000.);
#27682=VECTOR('',#127408,1000.);
#27683=VECTOR('',#127413,10.);
#27684=VECTOR('',#127420,10.);
#27685=VECTOR('',#127423,1000.);
#27686=VECTOR('',#127426,1000.);
#27687=VECTOR('',#127455,1000.);
#27688=VECTOR('',#127462,1000.);
#27689=VECTOR('',#127465,10.);
#27690=VECTOR('',#127468,10.);
#27691=VECTOR('',#127473,1000.);
#27692=VECTOR('',#127476,1000.);
#27693=VECTOR('',#127481,10.);
#27694=VECTOR('',#127488,10.);
#27695=VECTOR('',#127491,1000.);
#27696=VECTOR('',#127494,1000.);
#27697=VECTOR('',#127523,1000.);
#27698=VECTOR('',#127530,1000.);
#27699=VECTOR('',#127533,10.);
#27700=VECTOR('',#127536,10.);
#27701=VECTOR('',#127541,1000.);
#27702=VECTOR('',#127544,1000.);
#27703=VECTOR('',#127549,10.);
#27704=VECTOR('',#127556,10.);
#27705=VECTOR('',#127559,1000.);
#27706=VECTOR('',#127562,1000.);
#27707=VECTOR('',#127591,1000.);
#27708=VECTOR('',#127598,1000.);
#27709=VECTOR('',#127601,10.);
#27710=VECTOR('',#127604,10.);
#27711=VECTOR('',#127609,1000.);
#27712=VECTOR('',#127612,1000.);
#27713=VECTOR('',#127617,10.);
#27714=VECTOR('',#127624,10.);
#27715=VECTOR('',#127627,1000.);
#27716=VECTOR('',#127630,1000.);
#27717=VECTOR('',#127659,1000.);
#27718=VECTOR('',#127666,1000.);
#27719=VECTOR('',#127669,10.);
#27720=VECTOR('',#127672,10.);
#27721=VECTOR('',#127677,1000.);
#27722=VECTOR('',#127680,1000.);
#27723=VECTOR('',#127685,10.);
#27724=VECTOR('',#127692,10.);
#27725=VECTOR('',#127695,1000.);
#27726=VECTOR('',#127698,1000.);
#27727=VECTOR('',#127727,1000.);
#27728=VECTOR('',#127734,1000.);
#27729=VECTOR('',#127737,10.);
#27730=VECTOR('',#127740,10.);
#27731=VECTOR('',#127745,1000.);
#27732=VECTOR('',#127748,1000.);
#27733=VECTOR('',#127753,10.);
#27734=VECTOR('',#127760,10.);
#27735=VECTOR('',#127763,1000.);
#27736=VECTOR('',#127766,1000.);
#27737=VECTOR('',#127795,1000.);
#27738=VECTOR('',#127802,1000.);
#27739=VECTOR('',#127805,10.);
#27740=VECTOR('',#127808,10.);
#27741=VECTOR('',#127813,1000.);
#27742=VECTOR('',#127816,1000.);
#27743=VECTOR('',#127821,10.);
#27744=VECTOR('',#127828,10.);
#27745=VECTOR('',#127831,1000.);
#27746=VECTOR('',#127834,1000.);
#27747=VECTOR('',#127863,1000.);
#27748=VECTOR('',#127870,1000.);
#27749=VECTOR('',#127873,10.);
#27750=VECTOR('',#127876,10.);
#27751=VECTOR('',#127881,1000.);
#27752=VECTOR('',#127884,1000.);
#27753=VECTOR('',#127889,10.);
#27754=VECTOR('',#127896,10.);
#27755=VECTOR('',#127899,1000.);
#27756=VECTOR('',#127902,1000.);
#27757=VECTOR('',#127931,1000.);
#27758=VECTOR('',#127938,1000.);
#27759=VECTOR('',#127941,10.);
#27760=VECTOR('',#127944,10.);
#27761=VECTOR('',#127949,1000.);
#27762=VECTOR('',#127952,1000.);
#27763=VECTOR('',#127957,10.);
#27764=VECTOR('',#127964,10.);
#27765=VECTOR('',#127967,1000.);
#27766=VECTOR('',#127970,1000.);
#27767=VECTOR('',#127999,1000.);
#27768=VECTOR('',#128006,1000.);
#27769=VECTOR('',#128009,10.);
#27770=VECTOR('',#128012,10.);
#27771=VECTOR('',#128017,1000.);
#27772=VECTOR('',#128020,1000.);
#27773=VECTOR('',#128025,10.);
#27774=VECTOR('',#128032,10.);
#27775=VECTOR('',#128035,1000.);
#27776=VECTOR('',#128038,1000.);
#27777=VECTOR('',#128067,1000.);
#27778=VECTOR('',#128074,1000.);
#27779=VECTOR('',#128077,10.);
#27780=VECTOR('',#128080,10.);
#27781=VECTOR('',#128085,1000.);
#27782=VECTOR('',#128088,1000.);
#27783=VECTOR('',#128093,10.);
#27784=VECTOR('',#128100,10.);
#27785=VECTOR('',#128103,1000.);
#27786=VECTOR('',#128106,1000.);
#27787=VECTOR('',#128135,1000.);
#27788=VECTOR('',#128142,1000.);
#27789=VECTOR('',#128145,10.);
#27790=VECTOR('',#128148,10.);
#27791=VECTOR('',#128153,1000.);
#27792=VECTOR('',#128156,1000.);
#27793=VECTOR('',#128161,10.);
#27794=VECTOR('',#128168,10.);
#27795=VECTOR('',#128171,1000.);
#27796=VECTOR('',#128174,1000.);
#27797=VECTOR('',#128203,1000.);
#27798=VECTOR('',#128210,1000.);
#27799=VECTOR('',#128213,10.);
#27800=VECTOR('',#128216,10.);
#27801=VECTOR('',#128221,1000.);
#27802=VECTOR('',#128224,1000.);
#27803=VECTOR('',#128229,10.);
#27804=VECTOR('',#128236,10.);
#27805=VECTOR('',#128239,1000.);
#27806=VECTOR('',#128242,1000.);
#27807=VECTOR('',#128271,1000.);
#27808=VECTOR('',#128278,1000.);
#27809=VECTOR('',#128281,10.);
#27810=VECTOR('',#128284,10.);
#27811=VECTOR('',#128289,1000.);
#27812=VECTOR('',#128292,1000.);
#27813=VECTOR('',#128297,10.);
#27814=VECTOR('',#128304,10.);
#27815=VECTOR('',#128307,1000.);
#27816=VECTOR('',#128310,1000.);
#27817=VECTOR('',#128339,1000.);
#27818=VECTOR('',#128346,1000.);
#27819=VECTOR('',#128349,10.);
#27820=VECTOR('',#128352,10.);
#27821=VECTOR('',#128357,1000.);
#27822=VECTOR('',#128360,1000.);
#27823=VECTOR('',#128365,10.);
#27824=VECTOR('',#128372,10.);
#27825=VECTOR('',#128375,1000.);
#27826=VECTOR('',#128378,1000.);
#27827=VECTOR('',#128407,1000.);
#27828=VECTOR('',#128414,1000.);
#27829=VECTOR('',#128417,10.);
#27830=VECTOR('',#128420,10.);
#27831=VECTOR('',#128425,1000.);
#27832=VECTOR('',#128428,1000.);
#27833=VECTOR('',#128433,10.);
#27834=VECTOR('',#128440,10.);
#27835=VECTOR('',#128443,1000.);
#27836=VECTOR('',#128446,1000.);
#27837=VECTOR('',#128475,1000.);
#27838=VECTOR('',#128482,1000.);
#27839=VECTOR('',#128485,10.);
#27840=VECTOR('',#128488,10.);
#27841=VECTOR('',#128493,1000.);
#27842=VECTOR('',#128496,1000.);
#27843=VECTOR('',#128501,10.);
#27844=VECTOR('',#128508,10.);
#27845=VECTOR('',#128511,1000.);
#27846=VECTOR('',#128514,1000.);
#27847=VECTOR('',#128543,1000.);
#27848=VECTOR('',#128550,1000.);
#27849=VECTOR('',#128553,10.);
#27850=VECTOR('',#128556,10.);
#27851=VECTOR('',#128561,1000.);
#27852=VECTOR('',#128564,1000.);
#27853=VECTOR('',#128569,10.);
#27854=VECTOR('',#128576,10.);
#27855=VECTOR('',#128579,1000.);
#27856=VECTOR('',#128582,1000.);
#27857=VECTOR('',#128611,1000.);
#27858=VECTOR('',#128618,1000.);
#27859=VECTOR('',#128621,10.);
#27860=VECTOR('',#128624,10.);
#27861=VECTOR('',#128629,1000.);
#27862=VECTOR('',#128632,1000.);
#27863=VECTOR('',#128637,10.);
#27864=VECTOR('',#128644,10.);
#27865=VECTOR('',#128647,1000.);
#27866=VECTOR('',#128650,1000.);
#27867=VECTOR('',#128679,1000.);
#27868=VECTOR('',#128686,1000.);
#27869=VECTOR('',#128689,10.);
#27870=VECTOR('',#128692,10.);
#27871=VECTOR('',#128697,1000.);
#27872=VECTOR('',#128700,1000.);
#27873=VECTOR('',#128705,10.);
#27874=VECTOR('',#128712,10.);
#27875=VECTOR('',#128715,1000.);
#27876=VECTOR('',#128718,1000.);
#27877=VECTOR('',#128747,1000.);
#27878=VECTOR('',#128754,1000.);
#27879=VECTOR('',#128757,10.);
#27880=VECTOR('',#128760,10.);
#27881=VECTOR('',#128765,1000.);
#27882=VECTOR('',#128768,1000.);
#27883=VECTOR('',#128773,10.);
#27884=VECTOR('',#128780,10.);
#27885=VECTOR('',#128783,1000.);
#27886=VECTOR('',#128786,1000.);
#27887=VECTOR('',#128815,1000.);
#27888=VECTOR('',#128822,1000.);
#27889=VECTOR('',#128825,10.);
#27890=VECTOR('',#128828,10.);
#27891=VECTOR('',#128833,1000.);
#27892=VECTOR('',#128836,1000.);
#27893=VECTOR('',#128841,10.);
#27894=VECTOR('',#128848,10.);
#27895=VECTOR('',#128851,1000.);
#27896=VECTOR('',#128854,1000.);
#27897=VECTOR('',#128883,1000.);
#27898=VECTOR('',#128890,1000.);
#27899=VECTOR('',#128893,10.);
#27900=VECTOR('',#128896,10.);
#27901=VECTOR('',#128901,1000.);
#27902=VECTOR('',#128904,1000.);
#27903=VECTOR('',#128909,10.);
#27904=VECTOR('',#128916,10.);
#27905=VECTOR('',#128919,1000.);
#27906=VECTOR('',#128922,1000.);
#27907=VECTOR('',#128951,1000.);
#27908=VECTOR('',#128958,1000.);
#27909=VECTOR('',#128961,10.);
#27910=VECTOR('',#128964,10.);
#27911=VECTOR('',#128969,1000.);
#27912=VECTOR('',#128972,1000.);
#27913=VECTOR('',#128977,10.);
#27914=VECTOR('',#128984,10.);
#27915=VECTOR('',#128987,1000.);
#27916=VECTOR('',#128990,1000.);
#27917=VECTOR('',#129019,1000.);
#27918=VECTOR('',#129026,1000.);
#27919=VECTOR('',#129029,10.);
#27920=VECTOR('',#129032,10.);
#27921=VECTOR('',#129037,1000.);
#27922=VECTOR('',#129040,1000.);
#27923=VECTOR('',#129045,10.);
#27924=VECTOR('',#129052,10.);
#27925=VECTOR('',#129055,1000.);
#27926=VECTOR('',#129058,1000.);
#27927=VECTOR('',#129087,1000.);
#27928=VECTOR('',#129094,1000.);
#27929=VECTOR('',#129097,10.);
#27930=VECTOR('',#129100,10.);
#27931=VECTOR('',#129105,1000.);
#27932=VECTOR('',#129108,1000.);
#27933=VECTOR('',#129113,10.);
#27934=VECTOR('',#129120,10.);
#27935=VECTOR('',#129123,1000.);
#27936=VECTOR('',#129126,1000.);
#27937=VECTOR('',#129155,1000.);
#27938=VECTOR('',#129162,1000.);
#27939=VECTOR('',#129165,10.);
#27940=VECTOR('',#129168,10.);
#27941=VECTOR('',#129173,1000.);
#27942=VECTOR('',#129176,1000.);
#27943=VECTOR('',#129181,10.);
#27944=VECTOR('',#129188,10.);
#27945=VECTOR('',#129191,1000.);
#27946=VECTOR('',#129194,1000.);
#27947=VECTOR('',#129223,1000.);
#27948=VECTOR('',#129230,1000.);
#27949=VECTOR('',#129233,10.);
#27950=VECTOR('',#129236,10.);
#27951=VECTOR('',#129241,1000.);
#27952=VECTOR('',#129244,1000.);
#27953=VECTOR('',#129249,10.);
#27954=VECTOR('',#129256,10.);
#27955=VECTOR('',#129259,1000.);
#27956=VECTOR('',#129262,1000.);
#27957=VECTOR('',#129291,1000.);
#27958=VECTOR('',#129298,1000.);
#27959=VECTOR('',#129301,10.);
#27960=VECTOR('',#129304,10.);
#27961=VECTOR('',#129309,1000.);
#27962=VECTOR('',#129312,1000.);
#27963=VECTOR('',#129317,10.);
#27964=VECTOR('',#129324,10.);
#27965=VECTOR('',#129327,1000.);
#27966=VECTOR('',#129330,1000.);
#27967=VECTOR('',#129359,1000.);
#27968=VECTOR('',#129366,1000.);
#27969=VECTOR('',#129369,10.);
#27970=VECTOR('',#129372,10.);
#27971=VECTOR('',#129377,1000.);
#27972=VECTOR('',#129380,1000.);
#27973=VECTOR('',#129385,10.);
#27974=VECTOR('',#129392,10.);
#27975=VECTOR('',#129395,1000.);
#27976=VECTOR('',#129398,1000.);
#27977=VECTOR('',#129427,1000.);
#27978=VECTOR('',#129434,1000.);
#27979=VECTOR('',#129437,10.);
#27980=VECTOR('',#129440,10.);
#27981=VECTOR('',#129445,1000.);
#27982=VECTOR('',#129448,1000.);
#27983=VECTOR('',#129453,10.);
#27984=VECTOR('',#129460,10.);
#27985=VECTOR('',#129463,1000.);
#27986=VECTOR('',#129466,1000.);
#27987=VECTOR('',#129495,1000.);
#27988=VECTOR('',#129502,1000.);
#27989=VECTOR('',#129505,10.);
#27990=VECTOR('',#129508,10.);
#27991=VECTOR('',#129513,1000.);
#27992=VECTOR('',#129516,1000.);
#27993=VECTOR('',#129521,10.);
#27994=VECTOR('',#129528,10.);
#27995=VECTOR('',#129531,1000.);
#27996=VECTOR('',#129534,1000.);
#27997=VECTOR('',#129563,1000.);
#27998=VECTOR('',#129570,1000.);
#27999=VECTOR('',#129573,10.);
#28000=VECTOR('',#129576,10.);
#28001=VECTOR('',#129581,1000.);
#28002=VECTOR('',#129584,1000.);
#28003=VECTOR('',#129589,10.);
#28004=VECTOR('',#129596,10.);
#28005=VECTOR('',#129599,1000.);
#28006=VECTOR('',#129602,1000.);
#28007=VECTOR('',#129631,1000.);
#28008=VECTOR('',#129638,1000.);
#28009=VECTOR('',#129641,10.);
#28010=VECTOR('',#129644,10.);
#28011=VECTOR('',#129649,1000.);
#28012=VECTOR('',#129652,1000.);
#28013=VECTOR('',#129657,10.);
#28014=VECTOR('',#129664,10.);
#28015=VECTOR('',#129667,1000.);
#28016=VECTOR('',#129670,1000.);
#28017=VECTOR('',#129699,1000.);
#28018=VECTOR('',#129706,1000.);
#28019=VECTOR('',#129709,10.);
#28020=VECTOR('',#129712,10.);
#28021=VECTOR('',#129717,1000.);
#28022=VECTOR('',#129720,1000.);
#28023=VECTOR('',#129725,10.);
#28024=VECTOR('',#129732,10.);
#28025=VECTOR('',#129735,1000.);
#28026=VECTOR('',#129738,1000.);
#28027=VECTOR('',#129767,1000.);
#28028=VECTOR('',#129774,1000.);
#28029=VECTOR('',#129777,10.);
#28030=VECTOR('',#129780,10.);
#28031=VECTOR('',#129785,1000.);
#28032=VECTOR('',#129788,1000.);
#28033=VECTOR('',#129793,10.);
#28034=VECTOR('',#129800,10.);
#28035=VECTOR('',#129803,1000.);
#28036=VECTOR('',#129806,1000.);
#28037=VECTOR('',#129835,1000.);
#28038=VECTOR('',#129842,1000.);
#28039=VECTOR('',#129845,10.);
#28040=VECTOR('',#129848,10.);
#28041=VECTOR('',#129853,1000.);
#28042=VECTOR('',#129856,1000.);
#28043=VECTOR('',#129861,10.);
#28044=VECTOR('',#129868,10.);
#28045=VECTOR('',#129871,1000.);
#28046=VECTOR('',#129874,1000.);
#28047=VECTOR('',#129903,1000.);
#28048=VECTOR('',#129910,1000.);
#28049=VECTOR('',#129913,10.);
#28050=VECTOR('',#129916,10.);
#28051=VECTOR('',#129921,1000.);
#28052=VECTOR('',#129924,1000.);
#28053=VECTOR('',#129929,10.);
#28054=VECTOR('',#129936,10.);
#28055=VECTOR('',#129939,1000.);
#28056=VECTOR('',#129942,1000.);
#28057=VECTOR('',#129971,1000.);
#28058=VECTOR('',#129978,1000.);
#28059=VECTOR('',#129981,10.);
#28060=VECTOR('',#129984,10.);
#28061=VECTOR('',#129989,1000.);
#28062=VECTOR('',#129992,1000.);
#28063=VECTOR('',#129997,10.);
#28064=VECTOR('',#130004,10.);
#28065=VECTOR('',#130007,1000.);
#28066=VECTOR('',#130010,1000.);
#28067=VECTOR('',#130039,1000.);
#28068=VECTOR('',#130046,1000.);
#28069=VECTOR('',#130049,10.);
#28070=VECTOR('',#130052,10.);
#28071=VECTOR('',#130057,1000.);
#28072=VECTOR('',#130060,1000.);
#28073=VECTOR('',#130065,10.);
#28074=VECTOR('',#130072,10.);
#28075=VECTOR('',#130075,1000.);
#28076=VECTOR('',#130078,1000.);
#28077=VECTOR('',#130107,1000.);
#28078=VECTOR('',#130114,1000.);
#28079=VECTOR('',#130117,10.);
#28080=VECTOR('',#130120,10.);
#28081=VECTOR('',#130125,1000.);
#28082=VECTOR('',#130128,1000.);
#28083=VECTOR('',#130133,10.);
#28084=VECTOR('',#130140,10.);
#28085=VECTOR('',#130143,1000.);
#28086=VECTOR('',#130146,1000.);
#28087=VECTOR('',#130175,1000.);
#28088=VECTOR('',#130182,1000.);
#28089=VECTOR('',#130185,10.);
#28090=VECTOR('',#130188,10.);
#28091=VECTOR('',#130193,1000.);
#28092=VECTOR('',#130196,1000.);
#28093=VECTOR('',#130201,10.);
#28094=VECTOR('',#130208,10.);
#28095=VECTOR('',#130211,1000.);
#28096=VECTOR('',#130214,1000.);
#28097=VECTOR('',#130245,1000.);
#28098=VECTOR('',#130252,1000.);
#28099=VECTOR('',#130255,10.);
#28100=VECTOR('',#130258,10.);
#28101=VECTOR('',#130263,1000.);
#28102=VECTOR('',#130266,1000.);
#28103=VECTOR('',#130271,10.);
#28104=VECTOR('',#130278,10.);
#28105=VECTOR('',#130281,1000.);
#28106=VECTOR('',#130284,1000.);
#28107=VECTOR('',#130315,1000.);
#28108=VECTOR('',#130318,1000.);
#28109=VECTOR('',#130325,10.);
#28110=VECTOR('',#130326,1000.);
#28111=VECTOR('',#130327,10.);
#28112=VECTOR('',#130330,1000.);
#28113=VECTOR('',#130331,10.);
#28114=VECTOR('',#130334,1000.);
#28115=VECTOR('',#130337,10.);
#28116=VECTOR('',#130338,1000.);
#28117=VECTOR('',#130343,10.);
#28118=VECTOR('',#130344,1000.);
#28119=VECTOR('',#130345,10.);
#28120=VECTOR('',#130348,1000.);
#28121=VECTOR('',#130349,10.);
#28122=VECTOR('',#130352,1000.);
#28123=VECTOR('',#130355,10.);
#28124=VECTOR('',#130356,1000.);
#28125=VECTOR('',#130451,1000.);
#28126=VECTOR('',#130454,1000.);
#28127=VECTOR('',#130461,10.);
#28128=VECTOR('',#130462,1000.);
#28129=VECTOR('',#130463,10.);
#28130=VECTOR('',#130466,1000.);
#28131=VECTOR('',#130467,10.);
#28132=VECTOR('',#130470,1000.);
#28133=VECTOR('',#130473,10.);
#28134=VECTOR('',#130474,1000.);
#28135=VECTOR('',#130479,10.);
#28136=VECTOR('',#130480,1000.);
#28137=VECTOR('',#130481,10.);
#28138=VECTOR('',#130484,1000.);
#28139=VECTOR('',#130485,10.);
#28140=VECTOR('',#130488,1000.);
#28141=VECTOR('',#130491,10.);
#28142=VECTOR('',#130492,1000.);
#28143=VECTOR('',#130495,1000.);
#28144=VECTOR('',#130498,1000.);
#28145=VECTOR('',#130505,10.);
#28146=VECTOR('',#130506,1000.);
#28147=VECTOR('',#130507,10.);
#28148=VECTOR('',#130510,1000.);
#28149=VECTOR('',#130511,10.);
#28150=VECTOR('',#130514,1000.);
#28151=VECTOR('',#130517,10.);
#28152=VECTOR('',#130518,1000.);
#28153=VECTOR('',#130523,10.);
#28154=VECTOR('',#130524,1000.);
#28155=VECTOR('',#130525,10.);
#28156=VECTOR('',#130528,1000.);
#28157=VECTOR('',#130529,10.);
#28158=VECTOR('',#130532,1000.);
#28159=VECTOR('',#130535,10.);
#28160=VECTOR('',#130536,1000.);
#28161=VECTOR('',#130539,1000.);
#28162=VECTOR('',#130542,1000.);
#28163=VECTOR('',#130549,10.);
#28164=VECTOR('',#130550,1000.);
#28165=VECTOR('',#130551,10.);
#28166=VECTOR('',#130554,1000.);
#28167=VECTOR('',#130555,10.);
#28168=VECTOR('',#130558,1000.);
#28169=VECTOR('',#130561,10.);
#28170=VECTOR('',#130562,1000.);
#28171=VECTOR('',#130567,10.);
#28172=VECTOR('',#130568,1000.);
#28173=VECTOR('',#130569,10.);
#28174=VECTOR('',#130572,1000.);
#28175=VECTOR('',#130573,10.);
#28176=VECTOR('',#130576,1000.);
#28177=VECTOR('',#130579,10.);
#28178=VECTOR('',#130580,1000.);
#28179=VECTOR('',#130583,1000.);
#28180=VECTOR('',#130586,1000.);
#28181=VECTOR('',#130593,10.);
#28182=VECTOR('',#130594,1000.);
#28183=VECTOR('',#130595,10.);
#28184=VECTOR('',#130598,1000.);
#28185=VECTOR('',#130599,10.);
#28186=VECTOR('',#130602,1000.);
#28187=VECTOR('',#130605,10.);
#28188=VECTOR('',#130606,1000.);
#28189=VECTOR('',#130611,10.);
#28190=VECTOR('',#130612,1000.);
#28191=VECTOR('',#130613,10.);
#28192=VECTOR('',#130616,1000.);
#28193=VECTOR('',#130617,10.);
#28194=VECTOR('',#130620,1000.);
#28195=VECTOR('',#130623,10.);
#28196=VECTOR('',#130624,1000.);
#28197=VECTOR('',#130627,1000.);
#28198=VECTOR('',#130630,1000.);
#28199=VECTOR('',#130637,10.);
#28200=VECTOR('',#130638,1000.);
#28201=VECTOR('',#130639,10.);
#28202=VECTOR('',#130642,1000.);
#28203=VECTOR('',#130643,10.);
#28204=VECTOR('',#130646,1000.);
#28205=VECTOR('',#130649,10.);
#28206=VECTOR('',#130650,1000.);
#28207=VECTOR('',#130655,10.);
#28208=VECTOR('',#130656,1000.);
#28209=VECTOR('',#130657,10.);
#28210=VECTOR('',#130660,1000.);
#28211=VECTOR('',#130661,10.);
#28212=VECTOR('',#130664,1000.);
#28213=VECTOR('',#130667,10.);
#28214=VECTOR('',#130668,1000.);
#28215=VECTOR('',#130671,1000.);
#28216=VECTOR('',#130674,1000.);
#28217=VECTOR('',#130681,10.);
#28218=VECTOR('',#130682,1000.);
#28219=VECTOR('',#130683,10.);
#28220=VECTOR('',#130686,1000.);
#28221=VECTOR('',#130687,10.);
#28222=VECTOR('',#130690,1000.);
#28223=VECTOR('',#130693,10.);
#28224=VECTOR('',#130694,1000.);
#28225=VECTOR('',#130699,10.);
#28226=VECTOR('',#130700,1000.);
#28227=VECTOR('',#130701,10.);
#28228=VECTOR('',#130704,1000.);
#28229=VECTOR('',#130705,10.);
#28230=VECTOR('',#130708,1000.);
#28231=VECTOR('',#130711,10.);
#28232=VECTOR('',#130712,1000.);
#28233=VECTOR('',#130715,1000.);
#28234=VECTOR('',#130718,1000.);
#28235=VECTOR('',#130725,10.);
#28236=VECTOR('',#130726,1000.);
#28237=VECTOR('',#130727,10.);
#28238=VECTOR('',#130730,1000.);
#28239=VECTOR('',#130731,10.);
#28240=VECTOR('',#130734,1000.);
#28241=VECTOR('',#130737,10.);
#28242=VECTOR('',#130738,1000.);
#28243=VECTOR('',#130743,10.);
#28244=VECTOR('',#130744,1000.);
#28245=VECTOR('',#130745,10.);
#28246=VECTOR('',#130748,1000.);
#28247=VECTOR('',#130749,10.);
#28248=VECTOR('',#130752,1000.);
#28249=VECTOR('',#130755,10.);
#28250=VECTOR('',#130756,1000.);
#28251=VECTOR('',#130759,1000.);
#28252=VECTOR('',#130762,1000.);
#28253=VECTOR('',#130769,10.);
#28254=VECTOR('',#130770,1000.);
#28255=VECTOR('',#130771,10.);
#28256=VECTOR('',#130774,1000.);
#28257=VECTOR('',#130775,10.);
#28258=VECTOR('',#130778,1000.);
#28259=VECTOR('',#130781,10.);
#28260=VECTOR('',#130782,1000.);
#28261=VECTOR('',#130787,10.);
#28262=VECTOR('',#130788,1000.);
#28263=VECTOR('',#130789,10.);
#28264=VECTOR('',#130792,1000.);
#28265=VECTOR('',#130793,10.);
#28266=VECTOR('',#130796,1000.);
#28267=VECTOR('',#130799,10.);
#28268=VECTOR('',#130800,1000.);
#28269=VECTOR('',#130803,1000.);
#28270=VECTOR('',#130806,1000.);
#28271=VECTOR('',#130813,10.);
#28272=VECTOR('',#130814,1000.);
#28273=VECTOR('',#130815,10.);
#28274=VECTOR('',#130818,1000.);
#28275=VECTOR('',#130819,10.);
#28276=VECTOR('',#130822,1000.);
#28277=VECTOR('',#130825,10.);
#28278=VECTOR('',#130826,1000.);
#28279=VECTOR('',#130831,10.);
#28280=VECTOR('',#130832,1000.);
#28281=VECTOR('',#130833,10.);
#28282=VECTOR('',#130836,1000.);
#28283=VECTOR('',#130837,10.);
#28284=VECTOR('',#130840,1000.);
#28285=VECTOR('',#130843,10.);
#28286=VECTOR('',#130844,1000.);
#28287=VECTOR('',#130847,1000.);
#28288=VECTOR('',#130850,1000.);
#28289=VECTOR('',#130857,10.);
#28290=VECTOR('',#130858,1000.);
#28291=VECTOR('',#130859,10.);
#28292=VECTOR('',#130862,1000.);
#28293=VECTOR('',#130863,10.);
#28294=VECTOR('',#130866,1000.);
#28295=VECTOR('',#130869,10.);
#28296=VECTOR('',#130870,1000.);
#28297=VECTOR('',#130875,10.);
#28298=VECTOR('',#130876,1000.);
#28299=VECTOR('',#130877,10.);
#28300=VECTOR('',#130880,1000.);
#28301=VECTOR('',#130881,10.);
#28302=VECTOR('',#130884,1000.);
#28303=VECTOR('',#130887,10.);
#28304=VECTOR('',#130888,1000.);
#28305=VECTOR('',#130891,1000.);
#28306=VECTOR('',#130894,1000.);
#28307=VECTOR('',#130901,10.);
#28308=VECTOR('',#130902,1000.);
#28309=VECTOR('',#130903,10.);
#28310=VECTOR('',#130906,1000.);
#28311=VECTOR('',#130907,10.);
#28312=VECTOR('',#130910,1000.);
#28313=VECTOR('',#130913,10.);
#28314=VECTOR('',#130914,1000.);
#28315=VECTOR('',#130919,10.);
#28316=VECTOR('',#130920,1000.);
#28317=VECTOR('',#130921,10.);
#28318=VECTOR('',#130924,1000.);
#28319=VECTOR('',#130925,10.);
#28320=VECTOR('',#130928,1000.);
#28321=VECTOR('',#130931,10.);
#28322=VECTOR('',#130932,1000.);
#28323=VECTOR('',#130935,1000.);
#28324=VECTOR('',#130938,1000.);
#28325=VECTOR('',#130945,10.);
#28326=VECTOR('',#130946,1000.);
#28327=VECTOR('',#130947,10.);
#28328=VECTOR('',#130950,1000.);
#28329=VECTOR('',#130951,10.);
#28330=VECTOR('',#130954,1000.);
#28331=VECTOR('',#130957,10.);
#28332=VECTOR('',#130958,1000.);
#28333=VECTOR('',#130963,10.);
#28334=VECTOR('',#130964,1000.);
#28335=VECTOR('',#130965,10.);
#28336=VECTOR('',#130968,1000.);
#28337=VECTOR('',#130969,10.);
#28338=VECTOR('',#130972,1000.);
#28339=VECTOR('',#130975,10.);
#28340=VECTOR('',#130976,1000.);
#28341=VECTOR('',#130979,1000.);
#28342=VECTOR('',#130982,1000.);
#28343=VECTOR('',#130989,10.);
#28344=VECTOR('',#130990,1000.);
#28345=VECTOR('',#130991,10.);
#28346=VECTOR('',#130994,1000.);
#28347=VECTOR('',#130995,10.);
#28348=VECTOR('',#130998,1000.);
#28349=VECTOR('',#131001,10.);
#28350=VECTOR('',#131002,1000.);
#28351=VECTOR('',#131007,10.);
#28352=VECTOR('',#131008,1000.);
#28353=VECTOR('',#131009,10.);
#28354=VECTOR('',#131012,1000.);
#28355=VECTOR('',#131013,10.);
#28356=VECTOR('',#131016,1000.);
#28357=VECTOR('',#131019,10.);
#28358=VECTOR('',#131020,1000.);
#28359=VECTOR('',#131023,1000.);
#28360=VECTOR('',#131026,1000.);
#28361=VECTOR('',#131033,10.);
#28362=VECTOR('',#131034,1000.);
#28363=VECTOR('',#131035,10.);
#28364=VECTOR('',#131038,1000.);
#28365=VECTOR('',#131039,10.);
#28366=VECTOR('',#131042,1000.);
#28367=VECTOR('',#131045,10.);
#28368=VECTOR('',#131046,1000.);
#28369=VECTOR('',#131051,10.);
#28370=VECTOR('',#131052,1000.);
#28371=VECTOR('',#131053,10.);
#28372=VECTOR('',#131056,1000.);
#28373=VECTOR('',#131057,10.);
#28374=VECTOR('',#131060,1000.);
#28375=VECTOR('',#131063,10.);
#28376=VECTOR('',#131064,1000.);
#28377=VECTOR('',#131067,1000.);
#28378=VECTOR('',#131070,1000.);
#28379=VECTOR('',#131077,10.);
#28380=VECTOR('',#131078,1000.);
#28381=VECTOR('',#131079,10.);
#28382=VECTOR('',#131082,1000.);
#28383=VECTOR('',#131083,10.);
#28384=VECTOR('',#131086,1000.);
#28385=VECTOR('',#131089,10.);
#28386=VECTOR('',#131090,1000.);
#28387=VECTOR('',#131095,10.);
#28388=VECTOR('',#131096,1000.);
#28389=VECTOR('',#131097,10.);
#28390=VECTOR('',#131100,1000.);
#28391=VECTOR('',#131101,10.);
#28392=VECTOR('',#131104,1000.);
#28393=VECTOR('',#131107,10.);
#28394=VECTOR('',#131108,1000.);
#28395=VECTOR('',#131111,1000.);
#28396=VECTOR('',#131114,1000.);
#28397=VECTOR('',#131121,10.);
#28398=VECTOR('',#131122,1000.);
#28399=VECTOR('',#131123,10.);
#28400=VECTOR('',#131126,1000.);
#28401=VECTOR('',#131127,10.);
#28402=VECTOR('',#131130,1000.);
#28403=VECTOR('',#131133,10.);
#28404=VECTOR('',#131134,1000.);
#28405=VECTOR('',#131139,10.);
#28406=VECTOR('',#131140,1000.);
#28407=VECTOR('',#131141,10.);
#28408=VECTOR('',#131144,1000.);
#28409=VECTOR('',#131145,10.);
#28410=VECTOR('',#131148,1000.);
#28411=VECTOR('',#131151,10.);
#28412=VECTOR('',#131152,1000.);
#28413=VECTOR('',#131155,1000.);
#28414=VECTOR('',#131158,1000.);
#28415=VECTOR('',#131165,10.);
#28416=VECTOR('',#131166,1000.);
#28417=VECTOR('',#131167,10.);
#28418=VECTOR('',#131170,1000.);
#28419=VECTOR('',#131171,10.);
#28420=VECTOR('',#131174,1000.);
#28421=VECTOR('',#131177,10.);
#28422=VECTOR('',#131178,1000.);
#28423=VECTOR('',#131183,10.);
#28424=VECTOR('',#131184,1000.);
#28425=VECTOR('',#131185,10.);
#28426=VECTOR('',#131188,1000.);
#28427=VECTOR('',#131189,10.);
#28428=VECTOR('',#131192,1000.);
#28429=VECTOR('',#131195,10.);
#28430=VECTOR('',#131196,1000.);
#28431=VECTOR('',#131199,1000.);
#28432=VECTOR('',#131202,1000.);
#28433=VECTOR('',#131209,10.);
#28434=VECTOR('',#131210,1000.);
#28435=VECTOR('',#131211,10.);
#28436=VECTOR('',#131214,1000.);
#28437=VECTOR('',#131215,10.);
#28438=VECTOR('',#131218,1000.);
#28439=VECTOR('',#131221,10.);
#28440=VECTOR('',#131222,1000.);
#28441=VECTOR('',#131227,10.);
#28442=VECTOR('',#131228,1000.);
#28443=VECTOR('',#131229,10.);
#28444=VECTOR('',#131232,1000.);
#28445=VECTOR('',#131233,10.);
#28446=VECTOR('',#131236,1000.);
#28447=VECTOR('',#131239,10.);
#28448=VECTOR('',#131240,1000.);
#28449=VECTOR('',#131243,1000.);
#28450=VECTOR('',#131246,1000.);
#28451=VECTOR('',#131253,10.);
#28452=VECTOR('',#131254,1000.);
#28453=VECTOR('',#131255,10.);
#28454=VECTOR('',#131258,1000.);
#28455=VECTOR('',#131259,10.);
#28456=VECTOR('',#131262,1000.);
#28457=VECTOR('',#131265,10.);
#28458=VECTOR('',#131266,1000.);
#28459=VECTOR('',#131271,10.);
#28460=VECTOR('',#131272,1000.);
#28461=VECTOR('',#131273,10.);
#28462=VECTOR('',#131276,1000.);
#28463=VECTOR('',#131277,10.);
#28464=VECTOR('',#131280,1000.);
#28465=VECTOR('',#131283,10.);
#28466=VECTOR('',#131284,1000.);
#28467=VECTOR('',#131287,1000.);
#28468=VECTOR('',#131290,1000.);
#28469=VECTOR('',#131297,10.);
#28470=VECTOR('',#131298,1000.);
#28471=VECTOR('',#131299,10.);
#28472=VECTOR('',#131302,1000.);
#28473=VECTOR('',#131303,10.);
#28474=VECTOR('',#131306,1000.);
#28475=VECTOR('',#131309,10.);
#28476=VECTOR('',#131310,1000.);
#28477=VECTOR('',#131315,10.);
#28478=VECTOR('',#131316,1000.);
#28479=VECTOR('',#131317,10.);
#28480=VECTOR('',#131320,1000.);
#28481=VECTOR('',#131321,10.);
#28482=VECTOR('',#131324,1000.);
#28483=VECTOR('',#131327,10.);
#28484=VECTOR('',#131328,1000.);
#28485=VECTOR('',#131331,1000.);
#28486=VECTOR('',#131334,1000.);
#28487=VECTOR('',#131341,10.);
#28488=VECTOR('',#131342,1000.);
#28489=VECTOR('',#131343,10.);
#28490=VECTOR('',#131346,1000.);
#28491=VECTOR('',#131347,10.);
#28492=VECTOR('',#131350,1000.);
#28493=VECTOR('',#131353,10.);
#28494=VECTOR('',#131354,1000.);
#28495=VECTOR('',#131359,10.);
#28496=VECTOR('',#131360,1000.);
#28497=VECTOR('',#131361,10.);
#28498=VECTOR('',#131364,1000.);
#28499=VECTOR('',#131365,10.);
#28500=VECTOR('',#131368,1000.);
#28501=VECTOR('',#131371,10.);
#28502=VECTOR('',#131372,1000.);
#28503=VECTOR('',#131375,1000.);
#28504=VECTOR('',#131378,1000.);
#28505=VECTOR('',#131385,10.);
#28506=VECTOR('',#131386,1000.);
#28507=VECTOR('',#131387,10.);
#28508=VECTOR('',#131390,1000.);
#28509=VECTOR('',#131391,10.);
#28510=VECTOR('',#131394,1000.);
#28511=VECTOR('',#131397,10.);
#28512=VECTOR('',#131398,1000.);
#28513=VECTOR('',#131403,10.);
#28514=VECTOR('',#131404,1000.);
#28515=VECTOR('',#131405,10.);
#28516=VECTOR('',#131408,1000.);
#28517=VECTOR('',#131409,10.);
#28518=VECTOR('',#131412,1000.);
#28519=VECTOR('',#131415,10.);
#28520=VECTOR('',#131416,1000.);
#28521=VECTOR('',#131419,1000.);
#28522=VECTOR('',#131422,1000.);
#28523=VECTOR('',#131429,10.);
#28524=VECTOR('',#131430,1000.);
#28525=VECTOR('',#131431,10.);
#28526=VECTOR('',#131434,1000.);
#28527=VECTOR('',#131435,10.);
#28528=VECTOR('',#131438,1000.);
#28529=VECTOR('',#131441,10.);
#28530=VECTOR('',#131442,1000.);
#28531=VECTOR('',#131447,10.);
#28532=VECTOR('',#131448,1000.);
#28533=VECTOR('',#131449,10.);
#28534=VECTOR('',#131452,1000.);
#28535=VECTOR('',#131453,10.);
#28536=VECTOR('',#131456,1000.);
#28537=VECTOR('',#131459,10.);
#28538=VECTOR('',#131460,1000.);
#28539=VECTOR('',#131463,1000.);
#28540=VECTOR('',#131466,1000.);
#28541=VECTOR('',#131473,10.);
#28542=VECTOR('',#131474,1000.);
#28543=VECTOR('',#131475,10.);
#28544=VECTOR('',#131478,1000.);
#28545=VECTOR('',#131479,10.);
#28546=VECTOR('',#131482,1000.);
#28547=VECTOR('',#131485,10.);
#28548=VECTOR('',#131486,1000.);
#28549=VECTOR('',#131491,10.);
#28550=VECTOR('',#131492,1000.);
#28551=VECTOR('',#131493,10.);
#28552=VECTOR('',#131496,1000.);
#28553=VECTOR('',#131497,10.);
#28554=VECTOR('',#131500,1000.);
#28555=VECTOR('',#131503,10.);
#28556=VECTOR('',#131504,1000.);
#28557=VECTOR('',#131507,1000.);
#28558=VECTOR('',#131510,1000.);
#28559=VECTOR('',#131517,10.);
#28560=VECTOR('',#131518,1000.);
#28561=VECTOR('',#131519,10.);
#28562=VECTOR('',#131522,1000.);
#28563=VECTOR('',#131523,10.);
#28564=VECTOR('',#131526,1000.);
#28565=VECTOR('',#131529,10.);
#28566=VECTOR('',#131530,1000.);
#28567=VECTOR('',#131535,10.);
#28568=VECTOR('',#131536,1000.);
#28569=VECTOR('',#131537,10.);
#28570=VECTOR('',#131540,1000.);
#28571=VECTOR('',#131541,10.);
#28572=VECTOR('',#131544,1000.);
#28573=VECTOR('',#131547,10.);
#28574=VECTOR('',#131548,1000.);
#28575=VECTOR('',#131551,1000.);
#28576=VECTOR('',#131554,1000.);
#28577=VECTOR('',#131561,10.);
#28578=VECTOR('',#131562,1000.);
#28579=VECTOR('',#131563,10.);
#28580=VECTOR('',#131566,1000.);
#28581=VECTOR('',#131567,10.);
#28582=VECTOR('',#131570,1000.);
#28583=VECTOR('',#131573,10.);
#28584=VECTOR('',#131574,1000.);
#28585=VECTOR('',#131579,10.);
#28586=VECTOR('',#131580,1000.);
#28587=VECTOR('',#131581,10.);
#28588=VECTOR('',#131584,1000.);
#28589=VECTOR('',#131585,10.);
#28590=VECTOR('',#131588,1000.);
#28591=VECTOR('',#131591,10.);
#28592=VECTOR('',#131592,1000.);
#28593=VECTOR('',#131595,1000.);
#28594=VECTOR('',#131598,1000.);
#28595=VECTOR('',#131605,10.);
#28596=VECTOR('',#131606,1000.);
#28597=VECTOR('',#131607,10.);
#28598=VECTOR('',#131610,1000.);
#28599=VECTOR('',#131611,10.);
#28600=VECTOR('',#131614,1000.);
#28601=VECTOR('',#131617,10.);
#28602=VECTOR('',#131618,1000.);
#28603=VECTOR('',#131623,10.);
#28604=VECTOR('',#131624,1000.);
#28605=VECTOR('',#131625,10.);
#28606=VECTOR('',#131628,1000.);
#28607=VECTOR('',#131629,10.);
#28608=VECTOR('',#131632,1000.);
#28609=VECTOR('',#131635,10.);
#28610=VECTOR('',#131636,1000.);
#28611=VECTOR('',#131639,1000.);
#28612=VECTOR('',#131642,1000.);
#28613=VECTOR('',#131649,10.);
#28614=VECTOR('',#131650,1000.);
#28615=VECTOR('',#131651,10.);
#28616=VECTOR('',#131654,1000.);
#28617=VECTOR('',#131655,10.);
#28618=VECTOR('',#131658,1000.);
#28619=VECTOR('',#131661,10.);
#28620=VECTOR('',#131662,1000.);
#28621=VECTOR('',#131667,10.);
#28622=VECTOR('',#131668,1000.);
#28623=VECTOR('',#131669,10.);
#28624=VECTOR('',#131672,1000.);
#28625=VECTOR('',#131673,10.);
#28626=VECTOR('',#131676,1000.);
#28627=VECTOR('',#131679,10.);
#28628=VECTOR('',#131680,1000.);
#28629=VECTOR('',#131683,1000.);
#28630=VECTOR('',#131686,1000.);
#28631=VECTOR('',#131693,10.);
#28632=VECTOR('',#131694,1000.);
#28633=VECTOR('',#131695,10.);
#28634=VECTOR('',#131698,1000.);
#28635=VECTOR('',#131699,10.);
#28636=VECTOR('',#131702,1000.);
#28637=VECTOR('',#131705,10.);
#28638=VECTOR('',#131706,1000.);
#28639=VECTOR('',#131711,10.);
#28640=VECTOR('',#131712,1000.);
#28641=VECTOR('',#131713,10.);
#28642=VECTOR('',#131716,1000.);
#28643=VECTOR('',#131717,10.);
#28644=VECTOR('',#131720,1000.);
#28645=VECTOR('',#131723,10.);
#28646=VECTOR('',#131724,1000.);
#28647=VECTOR('',#131727,1000.);
#28648=VECTOR('',#131728,1000.);
#28649=VECTOR('',#131733,10.);
#28650=VECTOR('',#131734,1000.);
#28651=VECTOR('',#131735,10.);
#28652=VECTOR('',#131738,1000.);
#28653=VECTOR('',#131739,10.);
#28654=VECTOR('',#131742,1000.);
#28655=VECTOR('',#131745,10.);
#28656=VECTOR('',#131746,1000.);
#28657=VECTOR('',#131751,10.);
#28658=VECTOR('',#131752,1000.);
#28659=VECTOR('',#131753,10.);
#28660=VECTOR('',#131756,1000.);
#28661=VECTOR('',#131757,10.);
#28662=VECTOR('',#131760,1000.);
#28663=VECTOR('',#131763,10.);
#28664=VECTOR('',#131764,1000.);
#28665=VECTOR('',#131767,1000.);
#28666=VECTOR('',#131770,1000.);
#28667=VECTOR('',#131777,10.);
#28668=VECTOR('',#131778,1000.);
#28669=VECTOR('',#131779,10.);
#28670=VECTOR('',#131782,1000.);
#28671=VECTOR('',#131783,10.);
#28672=VECTOR('',#131786,1000.);
#28673=VECTOR('',#131789,10.);
#28674=VECTOR('',#131790,1000.);
#28675=VECTOR('',#131795,10.);
#28676=VECTOR('',#131796,1000.);
#28677=VECTOR('',#131797,10.);
#28678=VECTOR('',#131800,1000.);
#28679=VECTOR('',#131801,10.);
#28680=VECTOR('',#131804,1000.);
#28681=VECTOR('',#131807,10.);
#28682=VECTOR('',#131808,1000.);
#28683=VECTOR('',#131811,1000.);
#28684=VECTOR('',#131814,1000.);
#28685=VECTOR('',#131821,10.);
#28686=VECTOR('',#131822,1000.);
#28687=VECTOR('',#131823,10.);
#28688=VECTOR('',#131826,1000.);
#28689=VECTOR('',#131827,10.);
#28690=VECTOR('',#131830,1000.);
#28691=VECTOR('',#131833,10.);
#28692=VECTOR('',#131834,1000.);
#28693=VECTOR('',#131839,10.);
#28694=VECTOR('',#131840,1000.);
#28695=VECTOR('',#131841,10.);
#28696=VECTOR('',#131844,1000.);
#28697=VECTOR('',#131845,10.);
#28698=VECTOR('',#131848,1000.);
#28699=VECTOR('',#131851,10.);
#28700=VECTOR('',#131852,1000.);
#28701=VECTOR('',#131855,1000.);
#28702=VECTOR('',#131858,1000.);
#28703=VECTOR('',#131865,10.);
#28704=VECTOR('',#131866,1000.);
#28705=VECTOR('',#131867,10.);
#28706=VECTOR('',#131870,1000.);
#28707=VECTOR('',#131871,10.);
#28708=VECTOR('',#131874,1000.);
#28709=VECTOR('',#131877,10.);
#28710=VECTOR('',#131878,1000.);
#28711=VECTOR('',#131883,10.);
#28712=VECTOR('',#131884,1000.);
#28713=VECTOR('',#131885,10.);
#28714=VECTOR('',#131888,1000.);
#28715=VECTOR('',#131889,10.);
#28716=VECTOR('',#131892,1000.);
#28717=VECTOR('',#131895,10.);
#28718=VECTOR('',#131896,1000.);
#28719=VECTOR('',#131899,1000.);
#28720=VECTOR('',#131902,1000.);
#28721=VECTOR('',#131909,10.);
#28722=VECTOR('',#131910,1000.);
#28723=VECTOR('',#131911,10.);
#28724=VECTOR('',#131914,1000.);
#28725=VECTOR('',#131915,10.);
#28726=VECTOR('',#131918,1000.);
#28727=VECTOR('',#131921,10.);
#28728=VECTOR('',#131922,1000.);
#28729=VECTOR('',#131927,10.);
#28730=VECTOR('',#131928,1000.);
#28731=VECTOR('',#131929,10.);
#28732=VECTOR('',#131932,1000.);
#28733=VECTOR('',#131933,10.);
#28734=VECTOR('',#131936,1000.);
#28735=VECTOR('',#131939,10.);
#28736=VECTOR('',#131940,1000.);
#28737=VECTOR('',#131943,1000.);
#28738=VECTOR('',#131946,1000.);
#28739=VECTOR('',#131953,10.);
#28740=VECTOR('',#131954,1000.);
#28741=VECTOR('',#131955,10.);
#28742=VECTOR('',#131958,1000.);
#28743=VECTOR('',#131959,10.);
#28744=VECTOR('',#131962,1000.);
#28745=VECTOR('',#131965,10.);
#28746=VECTOR('',#131966,1000.);
#28747=VECTOR('',#131971,10.);
#28748=VECTOR('',#131972,1000.);
#28749=VECTOR('',#131973,10.);
#28750=VECTOR('',#131976,1000.);
#28751=VECTOR('',#131977,10.);
#28752=VECTOR('',#131980,1000.);
#28753=VECTOR('',#131983,10.);
#28754=VECTOR('',#131984,1000.);
#28755=VECTOR('',#131987,1000.);
#28756=VECTOR('',#131990,1000.);
#28757=VECTOR('',#131997,10.);
#28758=VECTOR('',#131998,1000.);
#28759=VECTOR('',#131999,10.);
#28760=VECTOR('',#132002,1000.);
#28761=VECTOR('',#132003,10.);
#28762=VECTOR('',#132006,1000.);
#28763=VECTOR('',#132009,10.);
#28764=VECTOR('',#132010,1000.);
#28765=VECTOR('',#132015,10.);
#28766=VECTOR('',#132016,1000.);
#28767=VECTOR('',#132017,10.);
#28768=VECTOR('',#132020,1000.);
#28769=VECTOR('',#132021,10.);
#28770=VECTOR('',#132024,1000.);
#28771=VECTOR('',#132027,10.);
#28772=VECTOR('',#132028,1000.);
#28773=VECTOR('',#132031,1000.);
#28774=VECTOR('',#132034,1000.);
#28775=VECTOR('',#132041,10.);
#28776=VECTOR('',#132042,1000.);
#28777=VECTOR('',#132043,10.);
#28778=VECTOR('',#132046,1000.);
#28779=VECTOR('',#132047,10.);
#28780=VECTOR('',#132050,1000.);
#28781=VECTOR('',#132053,10.);
#28782=VECTOR('',#132054,1000.);
#28783=VECTOR('',#132059,10.);
#28784=VECTOR('',#132060,1000.);
#28785=VECTOR('',#132061,10.);
#28786=VECTOR('',#132064,1000.);
#28787=VECTOR('',#132065,10.);
#28788=VECTOR('',#132068,1000.);
#28789=VECTOR('',#132071,10.);
#28790=VECTOR('',#132072,1000.);
#28791=VECTOR('',#132075,1000.);
#28792=VECTOR('',#132078,1000.);
#28793=VECTOR('',#132085,10.);
#28794=VECTOR('',#132086,1000.);
#28795=VECTOR('',#132087,10.);
#28796=VECTOR('',#132090,1000.);
#28797=VECTOR('',#132091,10.);
#28798=VECTOR('',#132094,1000.);
#28799=VECTOR('',#132097,10.);
#28800=VECTOR('',#132098,1000.);
#28801=VECTOR('',#132103,10.);
#28802=VECTOR('',#132104,1000.);
#28803=VECTOR('',#132105,10.);
#28804=VECTOR('',#132108,1000.);
#28805=VECTOR('',#132109,10.);
#28806=VECTOR('',#132112,1000.);
#28807=VECTOR('',#132115,10.);
#28808=VECTOR('',#132116,1000.);
#28809=VECTOR('',#132119,1000.);
#28810=VECTOR('',#132122,1000.);
#28811=VECTOR('',#132129,10.);
#28812=VECTOR('',#132130,1000.);
#28813=VECTOR('',#132131,10.);
#28814=VECTOR('',#132134,1000.);
#28815=VECTOR('',#132135,10.);
#28816=VECTOR('',#132138,1000.);
#28817=VECTOR('',#132141,10.);
#28818=VECTOR('',#132142,1000.);
#28819=VECTOR('',#132147,10.);
#28820=VECTOR('',#132148,1000.);
#28821=VECTOR('',#132149,10.);
#28822=VECTOR('',#132152,1000.);
#28823=VECTOR('',#132153,10.);
#28824=VECTOR('',#132156,1000.);
#28825=VECTOR('',#132159,10.);
#28826=VECTOR('',#132160,1000.);
#28827=VECTOR('',#132163,1000.);
#28828=VECTOR('',#132166,1000.);
#28829=VECTOR('',#132173,10.);
#28830=VECTOR('',#132174,1000.);
#28831=VECTOR('',#132175,10.);
#28832=VECTOR('',#132178,1000.);
#28833=VECTOR('',#132179,10.);
#28834=VECTOR('',#132182,1000.);
#28835=VECTOR('',#132185,10.);
#28836=VECTOR('',#132186,1000.);
#28837=VECTOR('',#132191,10.);
#28838=VECTOR('',#132192,1000.);
#28839=VECTOR('',#132193,10.);
#28840=VECTOR('',#132196,1000.);
#28841=VECTOR('',#132197,10.);
#28842=VECTOR('',#132200,1000.);
#28843=VECTOR('',#132203,10.);
#28844=VECTOR('',#132204,1000.);
#28845=VECTOR('',#132207,1000.);
#28846=VECTOR('',#132210,1000.);
#28847=VECTOR('',#132217,10.);
#28848=VECTOR('',#132218,1000.);
#28849=VECTOR('',#132219,10.);
#28850=VECTOR('',#132222,1000.);
#28851=VECTOR('',#132223,10.);
#28852=VECTOR('',#132226,1000.);
#28853=VECTOR('',#132229,10.);
#28854=VECTOR('',#132230,1000.);
#28855=VECTOR('',#132235,10.);
#28856=VECTOR('',#132236,1000.);
#28857=VECTOR('',#132237,10.);
#28858=VECTOR('',#132240,1000.);
#28859=VECTOR('',#132241,10.);
#28860=VECTOR('',#132244,1000.);
#28861=VECTOR('',#132247,10.);
#28862=VECTOR('',#132248,1000.);
#28863=VECTOR('',#132251,1000.);
#28864=VECTOR('',#132254,1000.);
#28865=VECTOR('',#132261,10.);
#28866=VECTOR('',#132262,1000.);
#28867=VECTOR('',#132263,10.);
#28868=VECTOR('',#132266,1000.);
#28869=VECTOR('',#132267,10.);
#28870=VECTOR('',#132270,1000.);
#28871=VECTOR('',#132273,10.);
#28872=VECTOR('',#132274,1000.);
#28873=VECTOR('',#132279,10.);
#28874=VECTOR('',#132280,1000.);
#28875=VECTOR('',#132281,10.);
#28876=VECTOR('',#132284,1000.);
#28877=VECTOR('',#132285,10.);
#28878=VECTOR('',#132288,1000.);
#28879=VECTOR('',#132291,10.);
#28880=VECTOR('',#132292,1000.);
#28881=VECTOR('',#132295,1000.);
#28882=VECTOR('',#132298,1000.);
#28883=VECTOR('',#132305,10.);
#28884=VECTOR('',#132306,1000.);
#28885=VECTOR('',#132307,10.);
#28886=VECTOR('',#132310,1000.);
#28887=VECTOR('',#132311,10.);
#28888=VECTOR('',#132314,1000.);
#28889=VECTOR('',#132317,10.);
#28890=VECTOR('',#132318,1000.);
#28891=VECTOR('',#132323,10.);
#28892=VECTOR('',#132324,1000.);
#28893=VECTOR('',#132325,10.);
#28894=VECTOR('',#132328,1000.);
#28895=VECTOR('',#132329,10.);
#28896=VECTOR('',#132332,1000.);
#28897=VECTOR('',#132335,10.);
#28898=VECTOR('',#132336,1000.);
#28899=VECTOR('',#132339,1000.);
#28900=VECTOR('',#132342,1000.);
#28901=VECTOR('',#132349,10.);
#28902=VECTOR('',#132350,1000.);
#28903=VECTOR('',#132351,10.);
#28904=VECTOR('',#132354,1000.);
#28905=VECTOR('',#132355,10.);
#28906=VECTOR('',#132358,1000.);
#28907=VECTOR('',#132361,10.);
#28908=VECTOR('',#132362,1000.);
#28909=VECTOR('',#132367,10.);
#28910=VECTOR('',#132368,1000.);
#28911=VECTOR('',#132369,10.);
#28912=VECTOR('',#132372,1000.);
#28913=VECTOR('',#132373,10.);
#28914=VECTOR('',#132376,1000.);
#28915=VECTOR('',#132379,10.);
#28916=VECTOR('',#132380,1000.);
#28917=VECTOR('',#132383,1000.);
#28918=VECTOR('',#132384,1000.);
#28919=VECTOR('',#132389,10.);
#28920=VECTOR('',#132390,1000.);
#28921=VECTOR('',#132391,10.);
#28922=VECTOR('',#132394,1000.);
#28923=VECTOR('',#132395,10.);
#28924=VECTOR('',#132398,1000.);
#28925=VECTOR('',#132401,10.);
#28926=VECTOR('',#132402,1000.);
#28927=VECTOR('',#132407,10.);
#28928=VECTOR('',#132408,1000.);
#28929=VECTOR('',#132409,10.);
#28930=VECTOR('',#132412,1000.);
#28931=VECTOR('',#132413,10.);
#28932=VECTOR('',#132416,1000.);
#28933=VECTOR('',#132419,10.);
#28934=VECTOR('',#132420,1000.);
#28935=VECTOR('',#132423,1000.);
#28936=VECTOR('',#132426,1000.);
#28937=VECTOR('',#132433,10.);
#28938=VECTOR('',#132434,1000.);
#28939=VECTOR('',#132435,10.);
#28940=VECTOR('',#132438,1000.);
#28941=VECTOR('',#132439,10.);
#28942=VECTOR('',#132442,1000.);
#28943=VECTOR('',#132445,10.);
#28944=VECTOR('',#132446,1000.);
#28945=VECTOR('',#132451,10.);
#28946=VECTOR('',#132452,1000.);
#28947=VECTOR('',#132453,10.);
#28948=VECTOR('',#132456,1000.);
#28949=VECTOR('',#132457,10.);
#28950=VECTOR('',#132460,1000.);
#28951=VECTOR('',#132463,10.);
#28952=VECTOR('',#132464,1000.);
#28953=VECTOR('',#132467,1000.);
#28954=VECTOR('',#132470,1000.);
#28955=VECTOR('',#132477,10.);
#28956=VECTOR('',#132478,1000.);
#28957=VECTOR('',#132479,10.);
#28958=VECTOR('',#132482,1000.);
#28959=VECTOR('',#132483,10.);
#28960=VECTOR('',#132486,1000.);
#28961=VECTOR('',#132489,10.);
#28962=VECTOR('',#132490,1000.);
#28963=VECTOR('',#132495,10.);
#28964=VECTOR('',#132496,1000.);
#28965=VECTOR('',#132497,10.);
#28966=VECTOR('',#132500,1000.);
#28967=VECTOR('',#132501,10.);
#28968=VECTOR('',#132504,1000.);
#28969=VECTOR('',#132507,10.);
#28970=VECTOR('',#132508,1000.);
#28971=VECTOR('',#132511,1000.);
#28972=VECTOR('',#132514,1000.);
#28973=VECTOR('',#132521,10.);
#28974=VECTOR('',#132522,1000.);
#28975=VECTOR('',#132523,10.);
#28976=VECTOR('',#132526,1000.);
#28977=VECTOR('',#132527,10.);
#28978=VECTOR('',#132530,1000.);
#28979=VECTOR('',#132533,10.);
#28980=VECTOR('',#132534,1000.);
#28981=VECTOR('',#132539,10.);
#28982=VECTOR('',#132540,1000.);
#28983=VECTOR('',#132541,10.);
#28984=VECTOR('',#132544,1000.);
#28985=VECTOR('',#132545,10.);
#28986=VECTOR('',#132548,1000.);
#28987=VECTOR('',#132551,10.);
#28988=VECTOR('',#132552,1000.);
#28989=VECTOR('',#132555,1000.);
#28990=VECTOR('',#132558,1000.);
#28991=VECTOR('',#132565,10.);
#28992=VECTOR('',#132566,1000.);
#28993=VECTOR('',#132567,10.);
#28994=VECTOR('',#132570,1000.);
#28995=VECTOR('',#132571,10.);
#28996=VECTOR('',#132574,1000.);
#28997=VECTOR('',#132577,10.);
#28998=VECTOR('',#132578,1000.);
#28999=VECTOR('',#132583,10.);
#29000=VECTOR('',#132584,1000.);
#29001=VECTOR('',#132585,10.);
#29002=VECTOR('',#132588,1000.);
#29003=VECTOR('',#132589,10.);
#29004=VECTOR('',#132592,1000.);
#29005=VECTOR('',#132595,10.);
#29006=VECTOR('',#132596,1000.);
#29007=VECTOR('',#132599,1000.);
#29008=VECTOR('',#132602,1000.);
#29009=VECTOR('',#132609,10.);
#29010=VECTOR('',#132610,1000.);
#29011=VECTOR('',#132611,10.);
#29012=VECTOR('',#132614,1000.);
#29013=VECTOR('',#132615,10.);
#29014=VECTOR('',#132618,1000.);
#29015=VECTOR('',#132621,10.);
#29016=VECTOR('',#132622,1000.);
#29017=VECTOR('',#132627,10.);
#29018=VECTOR('',#132628,1000.);
#29019=VECTOR('',#132629,10.);
#29020=VECTOR('',#132632,1000.);
#29021=VECTOR('',#132633,10.);
#29022=VECTOR('',#132636,1000.);
#29023=VECTOR('',#132639,10.);
#29024=VECTOR('',#132640,1000.);
#29025=VECTOR('',#132643,1000.);
#29026=VECTOR('',#132646,1000.);
#29027=VECTOR('',#132653,10.);
#29028=VECTOR('',#132654,1000.);
#29029=VECTOR('',#132655,10.);
#29030=VECTOR('',#132658,1000.);
#29031=VECTOR('',#132659,10.);
#29032=VECTOR('',#132662,1000.);
#29033=VECTOR('',#132665,10.);
#29034=VECTOR('',#132666,1000.);
#29035=VECTOR('',#132671,10.);
#29036=VECTOR('',#132672,1000.);
#29037=VECTOR('',#132673,10.);
#29038=VECTOR('',#132676,1000.);
#29039=VECTOR('',#132677,10.);
#29040=VECTOR('',#132680,1000.);
#29041=VECTOR('',#132683,10.);
#29042=VECTOR('',#132684,1000.);
#29043=VECTOR('',#132687,1000.);
#29044=VECTOR('',#132690,1000.);
#29045=VECTOR('',#132697,10.);
#29046=VECTOR('',#132698,1000.);
#29047=VECTOR('',#132699,10.);
#29048=VECTOR('',#132702,1000.);
#29049=VECTOR('',#132703,10.);
#29050=VECTOR('',#132706,1000.);
#29051=VECTOR('',#132709,10.);
#29052=VECTOR('',#132710,1000.);
#29053=VECTOR('',#132715,10.);
#29054=VECTOR('',#132716,1000.);
#29055=VECTOR('',#132717,10.);
#29056=VECTOR('',#132720,1000.);
#29057=VECTOR('',#132721,10.);
#29058=VECTOR('',#132724,1000.);
#29059=VECTOR('',#132727,10.);
#29060=VECTOR('',#132728,1000.);
#29061=VECTOR('',#132731,1000.);
#29062=VECTOR('',#132734,1000.);
#29063=VECTOR('',#132741,10.);
#29064=VECTOR('',#132742,1000.);
#29065=VECTOR('',#132743,10.);
#29066=VECTOR('',#132746,1000.);
#29067=VECTOR('',#132747,10.);
#29068=VECTOR('',#132750,1000.);
#29069=VECTOR('',#132753,10.);
#29070=VECTOR('',#132754,1000.);
#29071=VECTOR('',#132759,10.);
#29072=VECTOR('',#132760,1000.);
#29073=VECTOR('',#132761,10.);
#29074=VECTOR('',#132764,1000.);
#29075=VECTOR('',#132765,10.);
#29076=VECTOR('',#132768,1000.);
#29077=VECTOR('',#132771,10.);
#29078=VECTOR('',#132772,1000.);
#29079=VECTOR('',#132775,1000.);
#29080=VECTOR('',#132778,1000.);
#29081=VECTOR('',#132785,10.);
#29082=VECTOR('',#132786,1000.);
#29083=VECTOR('',#132787,10.);
#29084=VECTOR('',#132790,1000.);
#29085=VECTOR('',#132791,10.);
#29086=VECTOR('',#132794,1000.);
#29087=VECTOR('',#132797,10.);
#29088=VECTOR('',#132798,1000.);
#29089=VECTOR('',#132803,10.);
#29090=VECTOR('',#132804,1000.);
#29091=VECTOR('',#132805,10.);
#29092=VECTOR('',#132808,1000.);
#29093=VECTOR('',#132809,10.);
#29094=VECTOR('',#132812,1000.);
#29095=VECTOR('',#132815,10.);
#29096=VECTOR('',#132816,1000.);
#29097=VECTOR('',#132819,1000.);
#29098=VECTOR('',#132822,1000.);
#29099=VECTOR('',#132829,10.);
#29100=VECTOR('',#132830,1000.);
#29101=VECTOR('',#132831,10.);
#29102=VECTOR('',#132834,1000.);
#29103=VECTOR('',#132835,10.);
#29104=VECTOR('',#132838,1000.);
#29105=VECTOR('',#132841,10.);
#29106=VECTOR('',#132842,1000.);
#29107=VECTOR('',#132847,10.);
#29108=VECTOR('',#132848,1000.);
#29109=VECTOR('',#132849,10.);
#29110=VECTOR('',#132852,1000.);
#29111=VECTOR('',#132853,10.);
#29112=VECTOR('',#132856,1000.);
#29113=VECTOR('',#132859,10.);
#29114=VECTOR('',#132860,1000.);
#29115=VECTOR('',#132863,1000.);
#29116=VECTOR('',#132866,1000.);
#29117=VECTOR('',#132873,10.);
#29118=VECTOR('',#132874,1000.);
#29119=VECTOR('',#132875,10.);
#29120=VECTOR('',#132878,1000.);
#29121=VECTOR('',#132879,10.);
#29122=VECTOR('',#132882,1000.);
#29123=VECTOR('',#132885,10.);
#29124=VECTOR('',#132886,1000.);
#29125=VECTOR('',#132891,10.);
#29126=VECTOR('',#132892,1000.);
#29127=VECTOR('',#132893,10.);
#29128=VECTOR('',#132896,1000.);
#29129=VECTOR('',#132897,10.);
#29130=VECTOR('',#132900,1000.);
#29131=VECTOR('',#132903,10.);
#29132=VECTOR('',#132904,1000.);
#29133=VECTOR('',#132907,1000.);
#29134=VECTOR('',#132910,1000.);
#29135=VECTOR('',#132917,10.);
#29136=VECTOR('',#132918,1000.);
#29137=VECTOR('',#132919,10.);
#29138=VECTOR('',#132922,1000.);
#29139=VECTOR('',#132923,10.);
#29140=VECTOR('',#132926,1000.);
#29141=VECTOR('',#132929,10.);
#29142=VECTOR('',#132930,1000.);
#29143=VECTOR('',#132935,10.);
#29144=VECTOR('',#132936,1000.);
#29145=VECTOR('',#132937,10.);
#29146=VECTOR('',#132940,1000.);
#29147=VECTOR('',#132941,10.);
#29148=VECTOR('',#132944,1000.);
#29149=VECTOR('',#132947,10.);
#29150=VECTOR('',#132948,1000.);
#29151=VECTOR('',#132951,1000.);
#29152=VECTOR('',#132954,1000.);
#29153=VECTOR('',#132961,10.);
#29154=VECTOR('',#132962,1000.);
#29155=VECTOR('',#132963,10.);
#29156=VECTOR('',#132966,1000.);
#29157=VECTOR('',#132967,10.);
#29158=VECTOR('',#132970,1000.);
#29159=VECTOR('',#132973,10.);
#29160=VECTOR('',#132974,1000.);
#29161=VECTOR('',#132979,10.);
#29162=VECTOR('',#132980,1000.);
#29163=VECTOR('',#132981,10.);
#29164=VECTOR('',#132984,1000.);
#29165=VECTOR('',#132985,10.);
#29166=VECTOR('',#132988,1000.);
#29167=VECTOR('',#132991,10.);
#29168=VECTOR('',#132992,1000.);
#29169=VECTOR('',#132995,1000.);
#29170=VECTOR('',#132998,1000.);
#29171=VECTOR('',#133005,10.);
#29172=VECTOR('',#133006,1000.);
#29173=VECTOR('',#133007,10.);
#29174=VECTOR('',#133010,1000.);
#29175=VECTOR('',#133011,10.);
#29176=VECTOR('',#133014,1000.);
#29177=VECTOR('',#133017,10.);
#29178=VECTOR('',#133018,1000.);
#29179=VECTOR('',#133023,10.);
#29180=VECTOR('',#133024,1000.);
#29181=VECTOR('',#133025,10.);
#29182=VECTOR('',#133028,1000.);
#29183=VECTOR('',#133029,10.);
#29184=VECTOR('',#133032,1000.);
#29185=VECTOR('',#133035,10.);
#29186=VECTOR('',#133036,1000.);
#29187=VECTOR('',#138471,65.254);
#29188=VECTOR('',#138474,68.75);
#29189=VECTOR('',#138479,72.53);
#29190=VECTOR('',#138508,65.);
#29191=VECTOR('',#138511,65.254);
#29192=VECTOR('',#138596,1000.);
#29193=VECTOR('',#138599,1000.);
#29194=VECTOR('',#138602,1000.);
#29195=VECTOR('',#138605,1000.);
#29196=VECTOR('',#138616,72.53);
#29197=VECTOR('',#138623,8.4455);
#29198=VECTOR('',#138630,8.4455);
#29199=VECTOR('',#138637,8.4455);
#29200=VECTOR('',#138644,8.4455);
#29201=VECTOR('',#138649,1000.);
#29202=VECTOR('',#138652,1000.);
#29203=VECTOR('',#138675,1000.);
#29204=VECTOR('',#138678,1000.);
#29205=VECTOR('',#138681,1000.);
#29206=VECTOR('',#138684,1000.);
#29207=VECTOR('',#138689,1000.);
#29208=VECTOR('',#138692,1000.);
#29209=VECTOR('',#138695,1000.);
#29210=VECTOR('',#138698,1000.);
#29211=VECTOR('',#138701,1000.);
#29212=VECTOR('',#138702,1000.);
#29213=VECTOR('',#138703,1000.);
#29214=VECTOR('',#138706,1000.);
#29215=VECTOR('',#138707,1000.);
#29216=VECTOR('',#138710,1000.);
#29217=VECTOR('',#138711,1000.);
#29218=VECTOR('',#138712,1000.);
#29219=VECTOR('',#138713,1000.);
#29220=VECTOR('',#138716,1000.);
#29221=VECTOR('',#138717,1000.);
#29222=VECTOR('',#138726,1000.);
#29223=VECTOR('',#138727,1000.);
#29224=VECTOR('',#138732,1000.);
#29225=VECTOR('',#138737,1000.);
#29226=VECTOR('',#138738,1000.);
#29227=VECTOR('',#138739,1000.);
#29228=VECTOR('',#138742,1000.);
#29229=VECTOR('',#138745,1000.);
#29230=VECTOR('',#138750,1000.);
#29231=VECTOR('',#138751,1000.);
#29232=VECTOR('',#138752,1000.);
#29233=VECTOR('',#138757,1000.);
#29234=VECTOR('',#138762,1000.);
#29235=VECTOR('',#138763,1000.);
#29236=VECTOR('',#138764,1000.);
#29237=VECTOR('',#138769,1000.);
#29238=VECTOR('',#138774,1000.);
#29239=VECTOR('',#138775,1000.);
#29240=VECTOR('',#138776,1000.);
#29241=VECTOR('',#138781,1000.);
#29242=VECTOR('',#138786,1000.);
#29243=VECTOR('',#138787,1000.);
#29244=VECTOR('',#138790,1000.);
#29245=VECTOR('',#138793,1000.);
#29246=VECTOR('',#138796,1000.);
#29247=VECTOR('',#138797,1000.);
#29248=VECTOR('',#138798,1000.);
#29249=VECTOR('',#138803,1000.);
#29250=VECTOR('',#138804,1000.);
#29251=VECTOR('',#138807,1000.);
#29252=VECTOR('',#138816,1000.);
#29253=VECTOR('',#138819,1000.);
#29254=VECTOR('',#138822,1000.);
#29255=VECTOR('',#138827,1000.);
#29256=VECTOR('',#138832,1000.);
#29257=VECTOR('',#138833,1000.);
#29258=VECTOR('',#138842,1000.);
#29259=VECTOR('',#138843,1000.);
#29260=VECTOR('',#138846,1000.);
#29261=VECTOR('',#138849,1000.);
#29262=VECTOR('',#138858,1000.);
#29263=VECTOR('',#138861,1000.);
#29264=VECTOR('',#138866,1000.);
#29265=VECTOR('',#138869,1000.);
#29266=VECTOR('',#138874,1000.);
#29267=VECTOR('',#138877,1000.);
#29268=VECTOR('',#138880,1000.);
#29269=VECTOR('',#138883,1000.);
#29270=VECTOR('',#138886,1000.);
#29271=VECTOR('',#138887,1000.);
#29272=VECTOR('',#138890,1000.);
#29273=VECTOR('',#138891,1000.);
#29274=VECTOR('',#138894,1000.);
#29275=VECTOR('',#138895,1000.);
#29276=VECTOR('',#138900,1000.);
#29277=VECTOR('',#138903,1000.);
#29278=VECTOR('',#138906,1000.);
#29279=VECTOR('',#138909,1000.);
#29280=VECTOR('',#138910,1000.);
#29281=VECTOR('',#138913,1000.);
#29282=VECTOR('',#138914,1000.);
#29283=VECTOR('',#138915,1000.);
#29284=VECTOR('',#138920,1000.);
#29285=VECTOR('',#138923,1000.);
#29286=VECTOR('',#138930,1000.);
#29287=VECTOR('',#138933,1000.);
#29288=VECTOR('',#138934,1000.);
#29289=VECTOR('',#138935,1000.);
#29290=VECTOR('',#138938,1000.);
#29291=VECTOR('',#138939,1000.);
#29292=VECTOR('',#138940,1000.);
#29293=VECTOR('',#138945,1000.);
#29294=VECTOR('',#138948,1000.);
#29295=VECTOR('',#138949,1000.);
#29296=VECTOR('',#138952,1000.);
#29297=VECTOR('',#138955,1000.);
#29298=VECTOR('',#138956,1000.);
#29299=VECTOR('',#139235,1.27);
#29300=VECTOR('',#139240,1.905);
#29301=VECTOR('',#139269,1.27);
#29302=VECTOR('',#139274,66.0995441972308);
#29303=VECTOR('',#139277,66.4805441972308);
#29304=VECTOR('',#139332,56.875);
#29305=VECTOR('',#139337,56.2993860673093);
#29306=VECTOR('',#139340,57.8669800961561);
#29307=VECTOR('',#139345,51.27);
#29308=VECTOR('',#139348,50.);
#29309=VECTOR('',#139355,65.);
#29310=VECTOR('',#139370,4.7227367061318);
#29311=VECTOR('',#139375,4.7227367061318);
#29312=VECTOR('',#139378,4.7227367061318);
#29313=VECTOR('',#139381,4.7227367061318);
#29314=VECTOR('',#139384,4.7227367061318);
#29315=VECTOR('',#139387,4.7227367061318);
#29316=VECTOR('',#139390,4.74980000000001);
#29317=VECTOR('',#139395,4.74980000000001);
#29318=VECTOR('',#139400,4.74980000000001);
#29319=VECTOR('',#139403,4.74980000000001);
#29320=VECTOR('',#139406,4.74980000000001);
#29321=VECTOR('',#139409,4.74980000000001);
#29322=VECTOR('',#139412,4.74980000000001);
#29323=VECTOR('',#139415,4.74980000000001);
#29324=VECTOR('',#139426,4.74980000000001);
#29325=VECTOR('',#139439,3.98780000000001);
#29326=VECTOR('',#139474,1000.);
#29327=VECTOR('',#139475,1000.);
#29328=VECTOR('',#139476,1000.);
#29329=VECTOR('',#139477,1000.);
#29330=VECTOR('',#139478,1000.);
#29331=VECTOR('',#139479,1000.);
#29332=VECTOR('',#139482,1000.);
#29333=VECTOR('',#139483,1000.);
#29334=VECTOR('',#139486,1000.);
#29335=VECTOR('',#139489,1000.);
#29336=VECTOR('',#139492,1000.);
#29337=VECTOR('',#139495,1000.);
#29338=VECTOR('',#139502,4.72273670613179);
#29339=VECTOR('',#139507,4.72273670613179);
#29340=VECTOR('',#139510,4.72273670613179);
#29341=VECTOR('',#139513,4.72273670613179);
#29342=VECTOR('',#139516,4.72273670613179);
#29343=VECTOR('',#139519,4.72273670613179);
#29344=VECTOR('',#139522,4.74980000000001);
#29345=VECTOR('',#139527,4.74980000000001);
#29346=VECTOR('',#139532,4.74980000000001);
#29347=VECTOR('',#139535,4.7498);
#29348=VECTOR('',#139538,4.7498);
#29349=VECTOR('',#139541,4.74980000000001);
#29350=VECTOR('',#139544,4.74980000000001);
#29351=VECTOR('',#139547,4.74980000000001);
#29352=VECTOR('',#139558,4.74980000000001);
#29353=VECTOR('',#139571,3.98780000000001);
#29354=VECTOR('',#139606,1000.);
#29355=VECTOR('',#139607,1000.);
#29356=VECTOR('',#139608,1000.);
#29357=VECTOR('',#139609,1000.);
#29358=VECTOR('',#139610,1000.);
#29359=VECTOR('',#139611,1000.);
#29360=VECTOR('',#139614,1000.);
#29361=VECTOR('',#139615,1000.);
#29362=VECTOR('',#139618,1000.);
#29363=VECTOR('',#139621,1000.);
#29364=VECTOR('',#139624,1000.);
#29365=VECTOR('',#139627,1000.);
#29366=VECTOR('',#139636,40.);
#29367=VECTOR('',#139645,40.);
#29368=VECTOR('',#139652,48.4864729374055);
#29369=VECTOR('',#139661,48.4864729374054);
#29370=VECTOR('',#139666,50.);
#29371=VECTOR('',#139667,50.);
#29372=VECTOR('',#139670,4.7625);
#29373=VECTOR('',#139673,4.7625);
#29374=VECTOR('',#139676,40.);
#29375=VECTOR('',#139677,40.);
#29376=VECTOR('',#139686,65.0000000000002);
#29377=VECTOR('',#139693,56.875);
#29378=VECTOR('',#139710,76.4577478255888);
#29379=VECTOR('',#139715,1000.);
#29380=VECTOR('',#139718,1000.);
#29381=VECTOR('',#139723,70.625);
#29382=VECTOR('',#139730,76.5847478255888);
#29383=VECTOR('',#139737,8.4455);
#29384=VECTOR('',#139744,8.4455);
#29385=VECTOR('',#139751,8.4455);
#29386=VECTOR('',#139758,8.4455);
#29387=VECTOR('',#139765,7.9375);
#29388=VECTOR('',#139772,7.9375);
#29389=VECTOR('',#139779,7.9375);
#29390=VECTOR('',#139786,7.9375);
#29391=VECTOR('',#139791,1000.);
#29392=VECTOR('',#139794,1000.);
#29393=VECTOR('',#139799,1000.);
#29394=VECTOR('',#139800,1000.);
#29395=VECTOR('',#139801,1000.);
#29396=VECTOR('',#139806,1000.);
#29397=VECTOR('',#139811,1000.);
#29398=VECTOR('',#139812,1000.);
#29399=VECTOR('',#139813,1000.);
#29400=VECTOR('',#139818,1000.);
#29401=VECTOR('',#139823,1000.);
#29402=VECTOR('',#139824,1000.);
#29403=VECTOR('',#139825,1000.);
#29404=VECTOR('',#139830,1000.);
#29405=VECTOR('',#139835,1000.);
#29406=VECTOR('',#139836,1000.);
#29407=VECTOR('',#139839,1000.);
#29408=VECTOR('',#139842,1000.);
#29409=VECTOR('',#139845,1000.);
#29410=VECTOR('',#139848,1000.);
#29411=VECTOR('',#139863,1000.);
#29412=VECTOR('',#139866,1000.);
#29413=VECTOR('',#139869,1000.);
#29414=VECTOR('',#139872,1000.);
#29415=VECTOR('',#139875,1000.);
#29416=VECTOR('',#139878,1000.);
#29417=VECTOR('',#139881,1000.);
#29418=VECTOR('',#139882,1000.);
#29419=VECTOR('',#139885,1000.);
#29420=VECTOR('',#139890,1000.);
#29421=VECTOR('',#139891,1000.);
#29422=VECTOR('',#139894,1000.);
#29423=VECTOR('',#139899,1000.);
#29424=VECTOR('',#139900,1000.);
#29425=VECTOR('',#139903,1000.);
#29426=VECTOR('',#139908,1000.);
#29427=VECTOR('',#139945,1000.);
#29428=VECTOR('',#139948,1000.);
#29429=VECTOR('',#139953,1000.);
#29430=VECTOR('',#139956,1000.);
#29431=VECTOR('',#139957,1000.);
#29432=VECTOR('',#139960,1000.);
#29433=VECTOR('',#139969,1000.);
#29434=VECTOR('',#139972,1000.);
#29435=VECTOR('',#139975,1000.);
#29436=VECTOR('',#139978,1000.);
#29437=VECTOR('',#139981,1000.);
#29438=VECTOR('',#139984,1000.);
#29439=VECTOR('',#139987,1000.);
#29440=VECTOR('',#139988,1000.);
#30456=CIRCLE('',#98941,2.94003217057229);
#30457=CIRCLE('',#98942,1.57226);
#30458=CIRCLE('',#98943,3.78554799125932);
#30459=CIRCLE('',#98944,3.78554799125932);
#30460=CIRCLE('',#98947,5.55625);
#30461=CIRCLE('',#98949,5.1435);
#30462=CIRCLE('',#98950,5.1435);
#30463=CIRCLE('',#98952,5.55625);
#30464=CIRCLE('',#98953,5.55625);
#30465=CIRCLE('',#98955,5.55625);
#30466=CIRCLE('',#98956,5.55625);
#30467=CIRCLE('',#98957,5.55625);
#30468=CIRCLE('',#98958,5.55625);
#30469=CIRCLE('',#98959,5.55625);
#30470=CIRCLE('',#98961,3.3479996643018);
#30471=CIRCLE('',#98963,3.31406494267269);
#30472=CIRCLE('',#98964,3.31406494267269);
#30473=CIRCLE('',#98965,0.635000000000008);
#30474=CIRCLE('',#98967,2.40973730802039);
#30475=CIRCLE('',#98968,2.40973730802039);
#30476=CIRCLE('',#98970,2.1119189867422);
#30477=CIRCLE('',#98971,0.317500000000003);
#30478=CIRCLE('',#98973,0.952499999999998);
#30479=CIRCLE('',#98974,0.952499999999998);
#30480=CIRCLE('',#98984,5.55625);
#30481=CIRCLE('',#98985,5.55625);
#30482=CIRCLE('',#98986,5.55625);
#30483=CIRCLE('',#98987,5.55625);
#30484=CIRCLE('',#98988,5.55625);
#30485=CIRCLE('',#99006,7.9375);
#30486=CIRCLE('',#99007,7.9375);
#30487=CIRCLE('',#99009,8.4455);
#30488=CIRCLE('',#99010,8.4455);
#30489=CIRCLE('',#99014,7.9375);
#30490=CIRCLE('',#99015,7.9375);
#30491=CIRCLE('',#99017,8.4455);
#30492=CIRCLE('',#99018,8.4455);
#30493=CIRCLE('',#99022,7.9375);
#30494=CIRCLE('',#99023,7.9375);
#30495=CIRCLE('',#99025,8.4455);
#30496=CIRCLE('',#99026,8.4455);
#30497=CIRCLE('',#99030,7.9375);
#30498=CIRCLE('',#99031,7.9375);
#30499=CIRCLE('',#99033,8.4455);
#30500=CIRCLE('',#99034,8.4455);
#30501=CIRCLE('',#99038,50.);
#30502=CIRCLE('',#99039,50.);
#30503=CIRCLE('',#99040,0.254);
#30504=CIRCLE('',#99041,50.254);
#30505=CIRCLE('',#99043,51.016);
#30506=CIRCLE('',#99044,0.254);
#30507=CIRCLE('',#99045,51.27);
#30508=CIRCLE('',#99046,51.27);
#30509=CIRCLE('',#99048,51.27);
#30510=CIRCLE('',#99050,50.);
#30511=CIRCLE('',#99054,56.621);
#30512=CIRCLE('',#99055,0.254);
#30513=CIRCLE('',#99056,56.875);
#30514=CIRCLE('',#99057,56.875);
#30515=CIRCLE('',#99059,55.605);
#30516=CIRCLE('',#99060,55.605);
#30517=CIRCLE('',#99061,0.254);
#30518=CIRCLE('',#99062,55.859);
#30519=CIRCLE('',#99064,56.875);
#30520=CIRCLE('',#99066,55.605);
#30521=CIRCLE('',#99070,51.27);
#30522=CIRCLE('',#99071,51.27);
#30523=CIRCLE('',#99073,55.605);
#30524=CIRCLE('',#99074,55.605);
#30525=CIRCLE('',#99078,59.0285554514622);
#30526=CIRCLE('',#99079,0.127000000000002);
#30527=CIRCLE('',#99080,58.9208533432504);
#30528=CIRCLE('',#99081,0.127000000000002);
#30529=CIRCLE('',#99083,62.9541466567496);
#30530=CIRCLE('',#99084,0.127000000000002);
#30531=CIRCLE('',#99085,62.8464445485378);
#30532=CIRCLE('',#99086,0.127000000000002);
#30533=CIRCLE('',#99088,59.0285554514622);
#30534=CIRCLE('',#99089,0.127000000000002);
#30535=CIRCLE('',#99090,58.9208533432504);
#30536=CIRCLE('',#99091,0.127000000000002);
#30537=CIRCLE('',#99093,62.9541466567496);
#30538=CIRCLE('',#99094,0.127000000000002);
#30539=CIRCLE('',#99095,62.8464445485378);
#30540=CIRCLE('',#99096,0.127000000000002);
#30541=CIRCLE('',#99097,62.9541466567496);
#30542=CIRCLE('',#99099,58.2189663438286);
#30543=CIRCLE('',#99100,0.635);
#30544=CIRCLE('',#99101,57.6804558027693);
#30545=CIRCLE('',#99102,57.6804558027693);
#30546=CIRCLE('',#99104,58.8470884664677);
#30547=CIRCLE('',#99105,0.635);
#30548=CIRCLE('',#99106,58.3085779254084);
#30549=CIRCLE('',#99108,63.5664220745916);
#30550=CIRCLE('',#99109,0.635);
#30551=CIRCLE('',#99110,63.0279115335323);
#30552=CIRCLE('',#99111,63.0279115335323);
#30553=CIRCLE('',#99113,64.1945441972308);
#30554=CIRCLE('',#99114,0.635);
#30555=CIRCLE('',#99115,63.6560336561714);
#30556=CIRCLE('',#99117,65.);
#30557=CIRCLE('',#99118,65.);
#30558=CIRCLE('',#99121,62.9541466567496);
#30559=CIRCLE('',#99122,62.4089800241499);
#30560=CIRCLE('',#99123,62.9541466567496);
#30561=CIRCLE('',#99124,62.4089800241499);
#30562=CIRCLE('',#99125,62.9541466567496);
#30563=CIRCLE('',#99126,62.4089800241499);
#30564=CIRCLE('',#99127,62.9541466567497);
#30565=CIRCLE('',#99128,62.4089800241499);
#30566=CIRCLE('',#99129,62.9541466567496);
#30567=CIRCLE('',#99130,62.4089800241499);
#30568=CIRCLE('',#99131,62.9541466567496);
#30569=CIRCLE('',#99132,62.4089800241499);
#30570=CIRCLE('',#99133,62.9541466567497);
#30571=CIRCLE('',#99134,62.4089800241499);
#30572=CIRCLE('',#99135,62.9541466567497);
#30573=CIRCLE('',#99136,62.4089800241499);
#30574=CIRCLE('',#99137,62.9541466567496);
#30575=CIRCLE('',#99138,62.4089800241499);
#30576=CIRCLE('',#99139,62.9541466567497);
#30577=CIRCLE('',#99140,62.4089800241499);
#30578=CIRCLE('',#99141,62.9541466567496);
#30579=CIRCLE('',#99142,62.4089800241499);
#30580=CIRCLE('',#99143,62.9541466567497);
#30581=CIRCLE('',#99144,62.4089800241499);
#30582=CIRCLE('',#99145,62.9541466567497);
#30583=CIRCLE('',#99146,62.4089800241499);
#30584=CIRCLE('',#99147,62.9541466567496);
#30585=CIRCLE('',#99148,62.4089800241499);
#30586=CIRCLE('',#99149,62.9541466567497);
#30587=CIRCLE('',#99150,62.4089800241499);
#30588=CIRCLE('',#99151,62.9541466567496);
#30589=CIRCLE('',#99152,62.4089800241499);
#30590=CIRCLE('',#99153,62.9541466567497);
#30591=CIRCLE('',#99154,62.4089800241499);
#30592=CIRCLE('',#99155,62.9541466567497);
#30593=CIRCLE('',#99156,62.4089800241499);
#30594=CIRCLE('',#99157,62.9541466567496);
#30595=CIRCLE('',#99158,62.4089800241499);
#30596=CIRCLE('',#99159,62.9541466567496);
#30597=CIRCLE('',#99160,62.4089800241499);
#30598=CIRCLE('',#99161,62.9541466567496);
#30599=CIRCLE('',#99162,62.4089800241499);
#30600=CIRCLE('',#99163,62.9541466567496);
#30601=CIRCLE('',#99164,62.4089800241499);
#30602=CIRCLE('',#99165,62.9541466567497);
#30603=CIRCLE('',#99166,62.4089800241499);
#30604=CIRCLE('',#99167,62.9541466567497);
#30605=CIRCLE('',#99168,62.4089800241499);
#30606=CIRCLE('',#99169,62.9541466567496);
#30607=CIRCLE('',#99170,62.4089800241499);
#30608=CIRCLE('',#99171,62.9541466567496);
#30609=CIRCLE('',#99172,62.4089800241499);
#30610=CIRCLE('',#99173,62.9541466567496);
#30611=CIRCLE('',#99174,62.4089800241499);
#30612=CIRCLE('',#99175,62.9541466567497);
#30613=CIRCLE('',#99176,62.4089800241499);
#30614=CIRCLE('',#99177,62.9541466567496);
#30615=CIRCLE('',#99178,62.4089800241499);
#30616=CIRCLE('',#99179,62.9541466567497);
#30617=CIRCLE('',#99180,62.4089800241499);
#30618=CIRCLE('',#99181,62.4089800241499);
#30619=CIRCLE('',#99182,62.9541466567497);
#30620=CIRCLE('',#99183,62.4089800241499);
#30621=CIRCLE('',#99184,62.9541466567496);
#30622=CIRCLE('',#99185,62.4089800241499);
#30623=CIRCLE('',#99186,62.9541466567496);
#30624=CIRCLE('',#99187,62.4089800241499);
#30625=CIRCLE('',#99188,62.9541466567496);
#30626=CIRCLE('',#99189,62.4089800241499);
#30627=CIRCLE('',#99190,62.9541466567497);
#30628=CIRCLE('',#99191,62.4089800241499);
#30629=CIRCLE('',#99192,62.9541466567496);
#30630=CIRCLE('',#99193,62.4089800241499);
#30631=CIRCLE('',#99194,62.9541466567497);
#30632=CIRCLE('',#99195,62.4089800241499);
#30633=CIRCLE('',#99196,62.9541466567497);
#30634=CIRCLE('',#99197,62.4089800241499);
#30635=CIRCLE('',#99198,62.9541466567497);
#30636=CIRCLE('',#99199,62.4089800241499);
#30637=CIRCLE('',#99200,62.9541466567496);
#30638=CIRCLE('',#99201,62.4089800241499);
#30639=CIRCLE('',#99202,62.9541466567496);
#30640=CIRCLE('',#99203,62.4089800241499);
#30641=CIRCLE('',#99204,62.9541466567496);
#30642=CIRCLE('',#99205,62.4089800241499);
#30643=CIRCLE('',#99206,62.9541466567497);
#30644=CIRCLE('',#99207,62.4089800241499);
#30645=CIRCLE('',#99208,62.9541466567496);
#30646=CIRCLE('',#99209,62.4089800241499);
#30647=CIRCLE('',#99210,62.4089800241499);
#30648=CIRCLE('',#99211,62.9541466567497);
#30649=CIRCLE('',#99212,62.4089800241499);
#30650=CIRCLE('',#99213,62.9541466567497);
#30651=CIRCLE('',#99214,62.4089800241499);
#30652=CIRCLE('',#99215,62.9541466567497);
#30653=CIRCLE('',#99216,62.4089800241499);
#30654=CIRCLE('',#99217,62.9541466567497);
#30655=CIRCLE('',#99218,62.4089800241499);
#30656=CIRCLE('',#99219,62.9541466567497);
#30657=CIRCLE('',#99220,62.4089800241499);
#30658=CIRCLE('',#99221,62.9541466567496);
#30659=CIRCLE('',#99222,62.4089800241499);
#30660=CIRCLE('',#99223,62.9541466567496);
#30661=CIRCLE('',#99224,62.4089800241499);
#30662=CIRCLE('',#99225,62.9541466567496);
#30663=CIRCLE('',#99226,62.4089800241499);
#30664=CIRCLE('',#99227,62.9541466567497);
#30665=CIRCLE('',#99228,62.4089800241499);
#30666=CIRCLE('',#99229,62.9541466567496);
#30667=CIRCLE('',#99230,62.4089800241499);
#30668=CIRCLE('',#99231,62.9541466567497);
#30669=CIRCLE('',#99232,62.4089800241499);
#30670=CIRCLE('',#99233,62.9541466567497);
#30671=CIRCLE('',#99234,62.4089800241499);
#30672=CIRCLE('',#99235,62.9541466567497);
#30673=CIRCLE('',#99236,62.4089800241499);
#30674=CIRCLE('',#99237,62.9541466567497);
#30675=CIRCLE('',#99238,62.4089800241499);
#30676=CIRCLE('',#99240,59.4660199758502);
#30677=CIRCLE('',#99241,58.9208533432504);
#30678=CIRCLE('',#99242,59.4660199758502);
#30679=CIRCLE('',#99243,58.9208533432504);
#30680=CIRCLE('',#99244,59.4660199758502);
#30681=CIRCLE('',#99245,58.9208533432504);
#30682=CIRCLE('',#99246,59.4660199758502);
#30683=CIRCLE('',#99247,58.9208533432504);
#30684=CIRCLE('',#99248,59.4660199758502);
#30685=CIRCLE('',#99249,58.9208533432504);
#30686=CIRCLE('',#99250,59.4660199758502);
#30687=CIRCLE('',#99251,58.9208533432504);
#30688=CIRCLE('',#99252,59.4660199758502);
#30689=CIRCLE('',#99253,58.9208533432504);
#30690=CIRCLE('',#99254,59.4660199758502);
#30691=CIRCLE('',#99255,58.9208533432504);
#30692=CIRCLE('',#99256,59.4660199758502);
#30693=CIRCLE('',#99257,58.9208533432504);
#30694=CIRCLE('',#99258,59.4660199758502);
#30695=CIRCLE('',#99259,58.9208533432504);
#30696=CIRCLE('',#99260,59.4660199758502);
#30697=CIRCLE('',#99261,58.9208533432504);
#30698=CIRCLE('',#99262,59.4660199758502);
#30699=CIRCLE('',#99263,58.9208533432504);
#30700=CIRCLE('',#99264,59.4660199758502);
#30701=CIRCLE('',#99265,58.9208533432504);
#30702=CIRCLE('',#99266,59.4660199758502);
#30703=CIRCLE('',#99267,58.9208533432504);
#30704=CIRCLE('',#99268,59.4660199758502);
#30705=CIRCLE('',#99269,58.9208533432504);
#30706=CIRCLE('',#99270,59.4660199758502);
#30707=CIRCLE('',#99271,58.9208533432504);
#30708=CIRCLE('',#99272,59.4660199758502);
#30709=CIRCLE('',#99273,58.9208533432504);
#30710=CIRCLE('',#99274,59.4660199758502);
#30711=CIRCLE('',#99275,58.9208533432504);
#30712=CIRCLE('',#99276,59.4660199758502);
#30713=CIRCLE('',#99277,58.9208533432504);
#30714=CIRCLE('',#99278,59.4660199758502);
#30715=CIRCLE('',#99279,58.9208533432504);
#30716=CIRCLE('',#99280,59.4660199758502);
#30717=CIRCLE('',#99281,58.9208533432504);
#30718=CIRCLE('',#99282,59.4660199758502);
#30719=CIRCLE('',#99283,58.9208533432504);
#30720=CIRCLE('',#99284,59.4660199758502);
#30721=CIRCLE('',#99285,58.9208533432504);
#30722=CIRCLE('',#99286,59.4660199758502);
#30723=CIRCLE('',#99287,58.9208533432504);
#30724=CIRCLE('',#99288,59.4660199758502);
#30725=CIRCLE('',#99289,58.9208533432504);
#30726=CIRCLE('',#99290,59.4660199758502);
#30727=CIRCLE('',#99291,58.9208533432504);
#30728=CIRCLE('',#99292,59.4660199758502);
#30729=CIRCLE('',#99293,58.9208533432504);
#30730=CIRCLE('',#99294,59.4660199758502);
#30731=CIRCLE('',#99295,58.9208533432504);
#30732=CIRCLE('',#99296,59.4660199758502);
#30733=CIRCLE('',#99297,58.9208533432504);
#30734=CIRCLE('',#99298,59.4660199758502);
#30735=CIRCLE('',#99299,58.9208533432504);
#30736=CIRCLE('',#99300,58.9208533432504);
#30737=CIRCLE('',#99301,59.4660199758502);
#30738=CIRCLE('',#99302,58.9208533432504);
#30739=CIRCLE('',#99303,59.4660199758502);
#30740=CIRCLE('',#99304,58.9208533432504);
#30741=CIRCLE('',#99305,59.4660199758502);
#30742=CIRCLE('',#99306,58.9208533432504);
#30743=CIRCLE('',#99307,59.4660199758502);
#30744=CIRCLE('',#99308,58.9208533432504);
#30745=CIRCLE('',#99309,59.4660199758502);
#30746=CIRCLE('',#99310,58.9208533432504);
#30747=CIRCLE('',#99311,59.4660199758502);
#30748=CIRCLE('',#99312,58.9208533432504);
#30749=CIRCLE('',#99313,59.4660199758502);
#30750=CIRCLE('',#99314,58.9208533432504);
#30751=CIRCLE('',#99315,59.4660199758502);
#30752=CIRCLE('',#99316,58.9208533432504);
#30753=CIRCLE('',#99317,59.4660199758502);
#30754=CIRCLE('',#99318,58.9208533432504);
#30755=CIRCLE('',#99319,59.4660199758502);
#30756=CIRCLE('',#99320,58.9208533432504);
#30757=CIRCLE('',#99321,59.4660199758502);
#30758=CIRCLE('',#99322,58.9208533432504);
#30759=CIRCLE('',#99323,59.4660199758502);
#30760=CIRCLE('',#99324,58.9208533432504);
#30761=CIRCLE('',#99325,59.4660199758502);
#30762=CIRCLE('',#99326,58.9208533432504);
#30763=CIRCLE('',#99327,59.4660199758502);
#30764=CIRCLE('',#99328,58.9208533432504);
#30765=CIRCLE('',#99329,59.4660199758502);
#30766=CIRCLE('',#99330,59.4660199758502);
#30767=CIRCLE('',#99331,58.9208533432504);
#30768=CIRCLE('',#99332,59.4660199758502);
#30769=CIRCLE('',#99333,58.9208533432504);
#30770=CIRCLE('',#99334,59.4660199758502);
#30771=CIRCLE('',#99335,58.9208533432504);
#30772=CIRCLE('',#99336,59.4660199758502);
#30773=CIRCLE('',#99337,58.9208533432504);
#30774=CIRCLE('',#99338,59.4660199758502);
#30775=CIRCLE('',#99339,58.9208533432504);
#30776=CIRCLE('',#99340,59.4660199758502);
#30777=CIRCLE('',#99341,58.9208533432504);
#30778=CIRCLE('',#99342,59.4660199758502);
#30779=CIRCLE('',#99343,58.9208533432504);
#30780=CIRCLE('',#99344,59.4660199758502);
#30781=CIRCLE('',#99345,58.9208533432504);
#30782=CIRCLE('',#99346,59.4660199758502);
#30783=CIRCLE('',#99347,58.9208533432504);
#30784=CIRCLE('',#99348,59.4660199758502);
#30785=CIRCLE('',#99349,58.9208533432504);
#30786=CIRCLE('',#99350,59.4660199758502);
#30787=CIRCLE('',#99351,58.9208533432504);
#30788=CIRCLE('',#99352,59.4660199758502);
#30789=CIRCLE('',#99353,58.9208533432504);
#30790=CIRCLE('',#99354,59.4660199758502);
#30791=CIRCLE('',#99355,58.9208533432504);
#30792=CIRCLE('',#99356,59.4660199758502);
#30793=CIRCLE('',#99357,58.9208533432504);
#30794=CIRCLE('',#99358,59.4660199758502);
#30795=CIRCLE('',#99360,56.875);
#30796=CIRCLE('',#99361,56.875);
#30797=CIRCLE('',#99363,56.875);
#30798=CIRCLE('',#99365,60.4792282238308);
#30799=CIRCLE('',#99366,60.0045305169095);
#30800=CIRCLE('',#99367,60.4792282238308);
#30801=CIRCLE('',#99368,60.4792282238308);
#30802=CIRCLE('',#99370,60.6419265158129);
#30803=CIRCLE('',#99372,61.0131030316259);
#30804=CIRCLE('',#99373,60.8618969683742);
#30805=CIRCLE('',#99375,61.3957717761693);
#30806=CIRCLE('',#99376,61.2330734841871);
#30807=CIRCLE('',#99377,61.3957717761693);
#30808=CIRCLE('',#99378,61.3957717761693);
#30809=CIRCLE('',#99380,61.8704694830905);
#30810=CIRCLE('',#99382,0.635007073208601);
#30811=CIRCLE('',#99383,0.635007073208629);
#30812=CIRCLE('',#99394,60.0045305169095);
#30813=CIRCLE('',#99395,60.4792282238308);
#30814=CIRCLE('',#99396,60.4792282238308);
#30815=CIRCLE('',#99397,60.4792282238308);
#30816=CIRCLE('',#99399,60.6419265158129);
#30817=CIRCLE('',#99401,60.8618969683742);
#30818=CIRCLE('',#99402,61.0131030316259);
#30819=CIRCLE('',#99404,61.2330734841871);
#30820=CIRCLE('',#99405,61.3957717761693);
#30821=CIRCLE('',#99406,61.3957717761693);
#30822=CIRCLE('',#99407,61.3957717761693);
#30823=CIRCLE('',#99409,61.8704694830905);
#30824=CIRCLE('',#99411,0.635007073208607);
#30825=CIRCLE('',#99412,0.635007073208605);
#30826=CIRCLE('',#99423,60.0045305169095);
#30827=CIRCLE('',#99424,60.4792282238308);
#30828=CIRCLE('',#99425,60.4792282238308);
#30829=CIRCLE('',#99426,60.4792282238308);
#30830=CIRCLE('',#99428,60.6419265158129);
#30831=CIRCLE('',#99430,60.8618969683742);
#30832=CIRCLE('',#99431,61.0131030316259);
#30833=CIRCLE('',#99433,61.2330734841871);
#30834=CIRCLE('',#99434,61.3957717761693);
#30835=CIRCLE('',#99435,61.3957717761693);
#30836=CIRCLE('',#99436,61.3957717761693);
#30837=CIRCLE('',#99438,61.8704694830905);
#30838=CIRCLE('',#99440,0.635007073208615);
#30839=CIRCLE('',#99441,0.635007073208627);
#30840=CIRCLE('',#99452,60.0045305169095);
#30841=CIRCLE('',#99453,60.4792282238308);
#30842=CIRCLE('',#99454,60.4792282238308);
#30843=CIRCLE('',#99455,60.4792282238308);
#30844=CIRCLE('',#99457,60.6419265158129);
#30845=CIRCLE('',#99459,60.8618969683742);
#30846=CIRCLE('',#99460,61.0131030316259);
#30847=CIRCLE('',#99462,61.2330734841871);
#30848=CIRCLE('',#99463,61.3957717761693);
#30849=CIRCLE('',#99464,61.3957717761693);
#30850=CIRCLE('',#99465,61.3957717761693);
#30851=CIRCLE('',#99467,61.8704694830905);
#30852=CIRCLE('',#99469,0.635007073208633);
#30853=CIRCLE('',#99470,0.635007073208601);
#30854=CIRCLE('',#99481,60.0045305169095);
#30855=CIRCLE('',#99482,60.4792282238308);
#30856=CIRCLE('',#99483,60.4792282238308);
#30857=CIRCLE('',#99484,60.4792282238308);
#30858=CIRCLE('',#99486,60.6419265158129);
#30859=CIRCLE('',#99488,60.8618969683742);
#30860=CIRCLE('',#99489,61.0131030316259);
#30861=CIRCLE('',#99491,61.2330734841871);
#30862=CIRCLE('',#99492,61.3957717761693);
#30863=CIRCLE('',#99493,61.3957717761693);
#30864=CIRCLE('',#99494,61.3957717761693);
#30865=CIRCLE('',#99496,61.8704694830905);
#30866=CIRCLE('',#99498,0.635007073208607);
#30867=CIRCLE('',#99499,0.635007073208594);
#30868=CIRCLE('',#99510,60.0045305169095);
#30869=CIRCLE('',#99511,60.4792282238308);
#30870=CIRCLE('',#99512,60.4792282238308);
#30871=CIRCLE('',#99513,60.4792282238308);
#30872=CIRCLE('',#99515,60.6419265158129);
#30873=CIRCLE('',#99517,60.8618969683742);
#30874=CIRCLE('',#99518,61.0131030316259);
#30875=CIRCLE('',#99520,61.2330734841871);
#30876=CIRCLE('',#99521,61.3957717761693);
#30877=CIRCLE('',#99522,61.3957717761693);
#30878=CIRCLE('',#99523,61.3957717761693);
#30879=CIRCLE('',#99525,61.8704694830905);
#30880=CIRCLE('',#99527,0.635007073208611);
#30881=CIRCLE('',#99528,0.635007073208602);
#30882=CIRCLE('',#99539,60.0045305169095);
#30883=CIRCLE('',#99540,60.4792282238308);
#30884=CIRCLE('',#99541,60.4792282238308);
#30885=CIRCLE('',#99542,60.4792282238308);
#30886=CIRCLE('',#99544,60.6419265158129);
#30887=CIRCLE('',#99546,60.8618969683742);
#30888=CIRCLE('',#99547,61.0131030316259);
#30889=CIRCLE('',#99549,61.2330734841871);
#30890=CIRCLE('',#99550,61.3957717761693);
#30891=CIRCLE('',#99551,61.3957717761693);
#30892=CIRCLE('',#99552,61.3957717761693);
#30893=CIRCLE('',#99554,61.8704694830905);
#30894=CIRCLE('',#99556,0.635007073208602);
#30895=CIRCLE('',#99557,0.635007073208613);
#30896=CIRCLE('',#99568,60.0045305169095);
#30897=CIRCLE('',#99569,60.4792282238308);
#30898=CIRCLE('',#99570,60.4792282238308);
#30899=CIRCLE('',#99571,60.4792282238308);
#30900=CIRCLE('',#99573,60.6419265158129);
#30901=CIRCLE('',#99575,60.8618969683742);
#30902=CIRCLE('',#99576,61.0131030316259);
#30903=CIRCLE('',#99578,61.2330734841871);
#30904=CIRCLE('',#99579,61.3957717761693);
#30905=CIRCLE('',#99580,61.3957717761693);
#30906=CIRCLE('',#99581,61.3957717761693);
#30907=CIRCLE('',#99583,61.8704694830905);
#30908=CIRCLE('',#99585,0.635007073208633);
#30909=CIRCLE('',#99586,0.635007073208603);
#30910=CIRCLE('',#99597,60.0045305169095);
#30911=CIRCLE('',#99598,60.4792282238308);
#30912=CIRCLE('',#99599,60.4792282238308);
#30913=CIRCLE('',#99600,60.4792282238308);
#30914=CIRCLE('',#99602,60.6419265158129);
#30915=CIRCLE('',#99604,60.8618969683742);
#30916=CIRCLE('',#99605,61.0131030316259);
#30917=CIRCLE('',#99607,61.2330734841871);
#30918=CIRCLE('',#99608,61.3957717761693);
#30919=CIRCLE('',#99609,61.3957717761693);
#30920=CIRCLE('',#99610,61.3957717761693);
#30921=CIRCLE('',#99612,61.8704694830905);
#30922=CIRCLE('',#99614,0.635007073208615);
#30923=CIRCLE('',#99615,0.635007073208628);
#30924=CIRCLE('',#99626,60.0045305169095);
#30925=CIRCLE('',#99627,60.4792282238308);
#30926=CIRCLE('',#99628,60.4792282238308);
#30927=CIRCLE('',#99629,60.4792282238308);
#30928=CIRCLE('',#99631,60.6419265158129);
#30929=CIRCLE('',#99633,60.8618969683742);
#30930=CIRCLE('',#99634,61.0131030316259);
#30931=CIRCLE('',#99636,61.2330734841871);
#30932=CIRCLE('',#99637,61.3957717761693);
#30933=CIRCLE('',#99638,61.3957717761693);
#30934=CIRCLE('',#99639,61.3957717761693);
#30935=CIRCLE('',#99641,61.8704694830905);
#30936=CIRCLE('',#99643,0.635007073208624);
#30937=CIRCLE('',#99644,0.635007073208631);
#30938=CIRCLE('',#99655,60.0045305169095);
#30939=CIRCLE('',#99656,60.4792282238308);
#30940=CIRCLE('',#99657,60.4792282238308);
#30941=CIRCLE('',#99658,60.4792282238308);
#30942=CIRCLE('',#99660,60.6419265158129);
#30943=CIRCLE('',#99662,60.8618969683742);
#30944=CIRCLE('',#99663,61.0131030316259);
#30945=CIRCLE('',#99665,61.2330734841871);
#30946=CIRCLE('',#99666,61.3957717761693);
#30947=CIRCLE('',#99667,61.3957717761693);
#30948=CIRCLE('',#99668,61.3957717761693);
#30949=CIRCLE('',#99670,61.8704694830905);
#30950=CIRCLE('',#99672,0.635007073208607);
#30951=CIRCLE('',#99673,0.635007073208634);
#30952=CIRCLE('',#99684,60.0045305169095);
#30953=CIRCLE('',#99685,60.4792282238308);
#30954=CIRCLE('',#99686,60.4792282238308);
#30955=CIRCLE('',#99687,60.4792282238308);
#30956=CIRCLE('',#99689,60.6419265158129);
#30957=CIRCLE('',#99691,60.8618969683742);
#30958=CIRCLE('',#99692,61.0131030316259);
#30959=CIRCLE('',#99694,61.2330734841871);
#30960=CIRCLE('',#99695,61.3957717761693);
#30961=CIRCLE('',#99696,61.3957717761693);
#30962=CIRCLE('',#99697,61.3957717761693);
#30963=CIRCLE('',#99699,61.8704694830905);
#30964=CIRCLE('',#99701,0.63500707320862);
#30965=CIRCLE('',#99702,0.635007073208639);
#30966=CIRCLE('',#99713,60.0045305169095);
#30967=CIRCLE('',#99714,60.4792282238308);
#30968=CIRCLE('',#99715,60.4792282238308);
#30969=CIRCLE('',#99716,60.4792282238308);
#30970=CIRCLE('',#99718,60.6419265158129);
#30971=CIRCLE('',#99720,60.8618969683742);
#30972=CIRCLE('',#99721,61.0131030316259);
#30973=CIRCLE('',#99723,61.2330734841871);
#30974=CIRCLE('',#99724,61.3957717761693);
#30975=CIRCLE('',#99725,61.3957717761693);
#30976=CIRCLE('',#99726,61.3957717761693);
#30977=CIRCLE('',#99728,61.8704694830905);
#30978=CIRCLE('',#99730,0.63500707320862);
#30979=CIRCLE('',#99731,0.635007073208627);
#30980=CIRCLE('',#99742,60.0045305169095);
#30981=CIRCLE('',#99743,60.4792282238308);
#30982=CIRCLE('',#99744,60.4792282238308);
#30983=CIRCLE('',#99745,60.4792282238308);
#30984=CIRCLE('',#99747,60.6419265158129);
#30985=CIRCLE('',#99749,60.8618969683742);
#30986=CIRCLE('',#99750,61.0131030316259);
#30987=CIRCLE('',#99752,61.2330734841871);
#30988=CIRCLE('',#99753,61.3957717761693);
#30989=CIRCLE('',#99754,61.3957717761693);
#30990=CIRCLE('',#99755,61.3957717761693);
#30991=CIRCLE('',#99757,61.8704694830905);
#30992=CIRCLE('',#99759,0.635007073208602);
#30993=CIRCLE('',#99760,0.635007073208611);
#30994=CIRCLE('',#99771,60.0045305169095);
#30995=CIRCLE('',#99772,60.4792282238308);
#30996=CIRCLE('',#99773,60.4792282238308);
#30997=CIRCLE('',#99774,60.4792282238308);
#30998=CIRCLE('',#99776,60.6419265158129);
#30999=CIRCLE('',#99778,60.8618969683742);
#31000=CIRCLE('',#99779,61.0131030316259);
#31001=CIRCLE('',#99781,61.2330734841871);
#31002=CIRCLE('',#99782,61.3957717761693);
#31003=CIRCLE('',#99783,61.3957717761693);
#31004=CIRCLE('',#99784,61.3957717761693);
#31005=CIRCLE('',#99786,61.8704694830905);
#31006=CIRCLE('',#99788,0.635007073208624);
#31007=CIRCLE('',#99789,0.635007073208605);
#31008=CIRCLE('',#99800,60.0045305169095);
#31009=CIRCLE('',#99801,60.4792282238308);
#31010=CIRCLE('',#99802,60.4792282238308);
#31011=CIRCLE('',#99803,60.4792282238308);
#31012=CIRCLE('',#99805,60.6419265158129);
#31013=CIRCLE('',#99807,60.8618969683742);
#31014=CIRCLE('',#99808,61.0131030316259);
#31015=CIRCLE('',#99810,61.2330734841871);
#31016=CIRCLE('',#99811,61.3957717761693);
#31017=CIRCLE('',#99812,61.3957717761693);
#31018=CIRCLE('',#99813,61.3957717761693);
#31019=CIRCLE('',#99815,61.8704694830905);
#31020=CIRCLE('',#99817,0.63500707320866);
#31021=CIRCLE('',#99818,0.635007073208591);
#31022=CIRCLE('',#99829,60.0045305169095);
#31023=CIRCLE('',#99830,60.4792282238308);
#31024=CIRCLE('',#99831,60.4792282238308);
#31025=CIRCLE('',#99832,60.4792282238308);
#31026=CIRCLE('',#99834,60.6419265158129);
#31027=CIRCLE('',#99836,60.8618969683742);
#31028=CIRCLE('',#99837,61.0131030316259);
#31029=CIRCLE('',#99839,61.2330734841871);
#31030=CIRCLE('',#99840,61.3957717761693);
#31031=CIRCLE('',#99841,61.3957717761693);
#31032=CIRCLE('',#99842,61.3957717761693);
#31033=CIRCLE('',#99844,61.8704694830905);
#31034=CIRCLE('',#99846,0.635007073208575);
#31035=CIRCLE('',#99847,0.635007073208613);
#31036=CIRCLE('',#99858,60.0045305169095);
#31037=CIRCLE('',#99859,60.4792282238308);
#31038=CIRCLE('',#99860,60.4792282238308);
#31039=CIRCLE('',#99861,60.4792282238308);
#31040=CIRCLE('',#99863,60.6419265158129);
#31041=CIRCLE('',#99865,60.8618969683742);
#31042=CIRCLE('',#99866,61.0131030316259);
#31043=CIRCLE('',#99868,61.2330734841871);
#31044=CIRCLE('',#99869,61.3957717761693);
#31045=CIRCLE('',#99870,61.3957717761693);
#31046=CIRCLE('',#99871,61.3957717761693);
#31047=CIRCLE('',#99873,61.8704694830905);
#31048=CIRCLE('',#99875,0.635007073208615);
#31049=CIRCLE('',#99876,0.635007073208595);
#31050=CIRCLE('',#99887,60.0045305169095);
#31051=CIRCLE('',#99888,60.4792282238308);
#31052=CIRCLE('',#99889,60.4792282238308);
#31053=CIRCLE('',#99890,60.4792282238308);
#31054=CIRCLE('',#99892,60.6419265158129);
#31055=CIRCLE('',#99894,60.8618969683742);
#31056=CIRCLE('',#99895,61.0131030316259);
#31057=CIRCLE('',#99897,61.2330734841871);
#31058=CIRCLE('',#99898,61.3957717761693);
#31059=CIRCLE('',#99899,61.3957717761693);
#31060=CIRCLE('',#99900,61.3957717761693);
#31061=CIRCLE('',#99902,61.8704694830905);
#31062=CIRCLE('',#99904,0.635007073208607);
#31063=CIRCLE('',#99905,0.635007073208594);
#31064=CIRCLE('',#99916,60.0045305169095);
#31065=CIRCLE('',#99917,60.4792282238308);
#31066=CIRCLE('',#99918,60.4792282238308);
#31067=CIRCLE('',#99919,60.4792282238308);
#31068=CIRCLE('',#99921,60.6419265158129);
#31069=CIRCLE('',#99923,60.8618969683742);
#31070=CIRCLE('',#99924,61.0131030316259);
#31071=CIRCLE('',#99926,61.2330734841871);
#31072=CIRCLE('',#99927,61.3957717761693);
#31073=CIRCLE('',#99928,61.3957717761693);
#31074=CIRCLE('',#99929,61.3957717761693);
#31075=CIRCLE('',#99931,61.8704694830905);
#31076=CIRCLE('',#99933,0.635007073208598);
#31077=CIRCLE('',#99934,0.635007073208625);
#31078=CIRCLE('',#99945,60.0045305169095);
#31079=CIRCLE('',#99946,60.4792282238308);
#31080=CIRCLE('',#99947,60.4792282238308);
#31081=CIRCLE('',#99948,60.4792282238308);
#31082=CIRCLE('',#99950,60.6419265158129);
#31083=CIRCLE('',#99952,60.8618969683742);
#31084=CIRCLE('',#99953,61.0131030316259);
#31085=CIRCLE('',#99955,61.2330734841871);
#31086=CIRCLE('',#99956,61.3957717761693);
#31087=CIRCLE('',#99957,61.3957717761693);
#31088=CIRCLE('',#99958,61.3957717761693);
#31089=CIRCLE('',#99960,61.8704694830905);
#31090=CIRCLE('',#99962,0.635007073208633);
#31091=CIRCLE('',#99963,0.635007073208599);
#31092=CIRCLE('',#99974,60.0045305169095);
#31093=CIRCLE('',#99975,60.4792282238308);
#31094=CIRCLE('',#99976,60.4792282238308);
#31095=CIRCLE('',#99977,60.4792282238308);
#31096=CIRCLE('',#99979,60.6419265158129);
#31097=CIRCLE('',#99981,60.8618969683742);
#31098=CIRCLE('',#99982,61.0131030316259);
#31099=CIRCLE('',#99984,61.2330734841871);
#31100=CIRCLE('',#99985,61.3957717761693);
#31101=CIRCLE('',#99986,61.3957717761693);
#31102=CIRCLE('',#99987,61.3957717761693);
#31103=CIRCLE('',#99989,61.8704694830905);
#31104=CIRCLE('',#99991,0.635007073208593);
#31105=CIRCLE('',#99992,0.635007073208574);
#31106=CIRCLE('',#100003,60.0045305169095);
#31107=CIRCLE('',#100004,60.4792282238308);
#31108=CIRCLE('',#100005,60.4792282238308);
#31109=CIRCLE('',#100006,60.4792282238308);
#31110=CIRCLE('',#100008,60.6419265158129);
#31111=CIRCLE('',#100010,60.8618969683742);
#31112=CIRCLE('',#100011,61.0131030316259);
#31113=CIRCLE('',#100013,61.2330734841871);
#31114=CIRCLE('',#100014,61.3957717761693);
#31115=CIRCLE('',#100015,61.3957717761693);
#31116=CIRCLE('',#100016,61.3957717761693);
#31117=CIRCLE('',#100018,61.8704694830905);
#31118=CIRCLE('',#100020,0.63500707320862);
#31119=CIRCLE('',#100021,0.63500707320863);
#31120=CIRCLE('',#100032,60.0045305169095);
#31121=CIRCLE('',#100033,60.4792282238308);
#31122=CIRCLE('',#100034,60.4792282238308);
#31123=CIRCLE('',#100035,60.4792282238308);
#31124=CIRCLE('',#100037,60.6419265158129);
#31125=CIRCLE('',#100039,60.8618969683742);
#31126=CIRCLE('',#100040,61.0131030316259);
#31127=CIRCLE('',#100042,61.2330734841871);
#31128=CIRCLE('',#100043,61.3957717761693);
#31129=CIRCLE('',#100044,61.3957717761693);
#31130=CIRCLE('',#100045,61.3957717761693);
#31131=CIRCLE('',#100047,61.8704694830905);
#31132=CIRCLE('',#100049,0.635007073208607);
#31133=CIRCLE('',#100050,0.635007073208609);
#31134=CIRCLE('',#100061,60.0045305169095);
#31135=CIRCLE('',#100062,60.4792282238308);
#31136=CIRCLE('',#100063,60.4792282238308);
#31137=CIRCLE('',#100064,60.4792282238308);
#31138=CIRCLE('',#100066,60.6419265158129);
#31139=CIRCLE('',#100068,60.8618969683742);
#31140=CIRCLE('',#100069,61.0131030316259);
#31141=CIRCLE('',#100071,61.2330734841871);
#31142=CIRCLE('',#100072,61.3957717761693);
#31143=CIRCLE('',#100073,61.3957717761693);
#31144=CIRCLE('',#100074,61.3957717761693);
#31145=CIRCLE('',#100076,61.8704694830905);
#31146=CIRCLE('',#100078,0.635007073208598);
#31147=CIRCLE('',#100079,0.635007073208644);
#31148=CIRCLE('',#100090,60.0045305169095);
#31149=CIRCLE('',#100091,60.4792282238308);
#31150=CIRCLE('',#100092,60.4792282238308);
#31151=CIRCLE('',#100093,60.4792282238308);
#31152=CIRCLE('',#100095,60.6419265158129);
#31153=CIRCLE('',#100097,60.8618969683742);
#31154=CIRCLE('',#100098,61.0131030316259);
#31155=CIRCLE('',#100100,61.2330734841871);
#31156=CIRCLE('',#100101,61.3957717761693);
#31157=CIRCLE('',#100102,61.3957717761693);
#31158=CIRCLE('',#100103,61.3957717761693);
#31159=CIRCLE('',#100105,61.8704694830905);
#31160=CIRCLE('',#100107,0.635007073208571);
#31161=CIRCLE('',#100108,0.635007073208592);
#31162=CIRCLE('',#100119,60.0045305169095);
#31163=CIRCLE('',#100120,60.4792282238308);
#31164=CIRCLE('',#100121,60.4792282238308);
#31165=CIRCLE('',#100122,60.4792282238308);
#31166=CIRCLE('',#100124,60.6419265158129);
#31167=CIRCLE('',#100126,60.8618969683742);
#31168=CIRCLE('',#100127,61.0131030316259);
#31169=CIRCLE('',#100129,61.2330734841871);
#31170=CIRCLE('',#100130,61.3957717761693);
#31171=CIRCLE('',#100131,61.3957717761693);
#31172=CIRCLE('',#100132,61.3957717761693);
#31173=CIRCLE('',#100134,61.8704694830905);
#31174=CIRCLE('',#100136,0.635007073208655);
#31175=CIRCLE('',#100137,0.635007073208618);
#31176=CIRCLE('',#100148,60.0045305169095);
#31177=CIRCLE('',#100149,60.4792282238308);
#31178=CIRCLE('',#100150,60.4792282238308);
#31179=CIRCLE('',#100151,60.4792282238308);
#31180=CIRCLE('',#100153,60.6419265158129);
#31181=CIRCLE('',#100155,60.8618969683742);
#31182=CIRCLE('',#100156,61.0131030316259);
#31183=CIRCLE('',#100158,61.2330734841871);
#31184=CIRCLE('',#100159,61.3957717761693);
#31185=CIRCLE('',#100160,61.3957717761693);
#31186=CIRCLE('',#100161,61.3957717761693);
#31187=CIRCLE('',#100163,61.8704694830905);
#31188=CIRCLE('',#100165,0.63500707320866);
#31189=CIRCLE('',#100166,0.635007073208662);
#31190=CIRCLE('',#100177,60.0045305169095);
#31191=CIRCLE('',#100178,60.4792282238308);
#31192=CIRCLE('',#100179,60.4792282238308);
#31193=CIRCLE('',#100180,60.4792282238308);
#31194=CIRCLE('',#100182,60.6419265158129);
#31195=CIRCLE('',#100184,60.8618969683742);
#31196=CIRCLE('',#100185,61.0131030316259);
#31197=CIRCLE('',#100187,61.2330734841871);
#31198=CIRCLE('',#100188,61.3957717761693);
#31199=CIRCLE('',#100189,61.3957717761693);
#31200=CIRCLE('',#100190,61.3957717761693);
#31201=CIRCLE('',#100192,61.8704694830905);
#31202=CIRCLE('',#100194,0.635007073208651);
#31203=CIRCLE('',#100195,0.635007073208644);
#31204=CIRCLE('',#100206,60.0045305169095);
#31205=CIRCLE('',#100207,60.4792282238308);
#31206=CIRCLE('',#100208,60.4792282238308);
#31207=CIRCLE('',#100209,60.4792282238308);
#31208=CIRCLE('',#100211,60.6419265158129);
#31209=CIRCLE('',#100213,60.8618969683742);
#31210=CIRCLE('',#100214,61.0131030316259);
#31211=CIRCLE('',#100216,61.2330734841871);
#31212=CIRCLE('',#100217,61.3957717761693);
#31213=CIRCLE('',#100218,61.3957717761693);
#31214=CIRCLE('',#100219,61.3957717761693);
#31215=CIRCLE('',#100221,61.8704694830905);
#31216=CIRCLE('',#100223,0.635007073208593);
#31217=CIRCLE('',#100224,0.635007073208605);
#31218=CIRCLE('',#100235,60.0045305169095);
#31219=CIRCLE('',#100236,60.4792282238308);
#31220=CIRCLE('',#100237,60.4792282238308);
#31221=CIRCLE('',#100238,60.4792282238308);
#31222=CIRCLE('',#100240,60.6419265158129);
#31223=CIRCLE('',#100242,60.8618969683742);
#31224=CIRCLE('',#100243,61.0131030316259);
#31225=CIRCLE('',#100245,61.2330734841871);
#31226=CIRCLE('',#100246,61.3957717761693);
#31227=CIRCLE('',#100247,61.3957717761693);
#31228=CIRCLE('',#100248,61.3957717761693);
#31229=CIRCLE('',#100250,61.8704694830905);
#31230=CIRCLE('',#100252,0.635007073208602);
#31231=CIRCLE('',#100253,0.63500707320862);
#31232=CIRCLE('',#100264,60.0045305169095);
#31233=CIRCLE('',#100265,60.4792282238308);
#31234=CIRCLE('',#100266,60.4792282238308);
#31235=CIRCLE('',#100267,60.4792282238308);
#31236=CIRCLE('',#100269,60.6419265158129);
#31237=CIRCLE('',#100271,60.8618969683742);
#31238=CIRCLE('',#100272,61.0131030316259);
#31239=CIRCLE('',#100274,61.2330734841871);
#31240=CIRCLE('',#100275,61.3957717761693);
#31241=CIRCLE('',#100276,61.3957717761693);
#31242=CIRCLE('',#100277,61.3957717761693);
#31243=CIRCLE('',#100279,61.8704694830905);
#31244=CIRCLE('',#100281,0.635007073208646);
#31245=CIRCLE('',#100282,0.635007073208569);
#31246=CIRCLE('',#100293,60.0045305169095);
#31247=CIRCLE('',#100294,60.4792282238308);
#31248=CIRCLE('',#100295,60.4792282238308);
#31249=CIRCLE('',#100296,60.4792282238308);
#31250=CIRCLE('',#100298,60.6419265158129);
#31251=CIRCLE('',#100300,60.8618969683742);
#31252=CIRCLE('',#100301,61.0131030316259);
#31253=CIRCLE('',#100303,61.2330734841871);
#31254=CIRCLE('',#100304,61.3957717761693);
#31255=CIRCLE('',#100305,61.3957717761693);
#31256=CIRCLE('',#100306,61.3957717761693);
#31257=CIRCLE('',#100308,61.8704694830905);
#31258=CIRCLE('',#100310,0.635007073208638);
#31259=CIRCLE('',#100311,0.63500707320862);
#31260=CIRCLE('',#100322,60.0045305169095);
#31261=CIRCLE('',#100323,60.4792282238308);
#31262=CIRCLE('',#100324,60.4792282238308);
#31263=CIRCLE('',#100325,60.4792282238308);
#31264=CIRCLE('',#100327,60.6419265158129);
#31265=CIRCLE('',#100329,60.8618969683742);
#31266=CIRCLE('',#100330,61.0131030316259);
#31267=CIRCLE('',#100332,61.2330734841871);
#31268=CIRCLE('',#100333,61.3957717761693);
#31269=CIRCLE('',#100334,61.3957717761693);
#31270=CIRCLE('',#100335,61.3957717761693);
#31271=CIRCLE('',#100337,61.8704694830905);
#31272=CIRCLE('',#100339,0.635007073208642);
#31273=CIRCLE('',#100340,0.635007073208594);
#31274=CIRCLE('',#100351,60.0045305169095);
#31275=CIRCLE('',#100352,60.4792282238308);
#31276=CIRCLE('',#100353,60.4792282238308);
#31277=CIRCLE('',#100354,60.4792282238308);
#31278=CIRCLE('',#100356,60.6419265158129);
#31279=CIRCLE('',#100358,60.8618969683742);
#31280=CIRCLE('',#100359,61.0131030316259);
#31281=CIRCLE('',#100361,61.2330734841871);
#31282=CIRCLE('',#100362,61.3957717761693);
#31283=CIRCLE('',#100363,61.3957717761693);
#31284=CIRCLE('',#100364,61.3957717761693);
#31285=CIRCLE('',#100366,61.8704694830905);
#31286=CIRCLE('',#100368,0.63500707320862);
#31287=CIRCLE('',#100369,0.635007073208609);
#31288=CIRCLE('',#100380,60.0045305169095);
#31289=CIRCLE('',#100381,60.4792282238308);
#31290=CIRCLE('',#100382,60.4792282238308);
#31291=CIRCLE('',#100383,60.4792282238308);
#31292=CIRCLE('',#100385,60.6419265158129);
#31293=CIRCLE('',#100387,60.8618969683742);
#31294=CIRCLE('',#100388,61.0131030316259);
#31295=CIRCLE('',#100390,61.2330734841871);
#31296=CIRCLE('',#100391,61.3957717761693);
#31297=CIRCLE('',#100392,61.3957717761693);
#31298=CIRCLE('',#100393,61.3957717761693);
#31299=CIRCLE('',#100395,61.8704694830905);
#31300=CIRCLE('',#100397,0.63500707320862);
#31301=CIRCLE('',#100398,0.635007073208601);
#31302=CIRCLE('',#100409,60.0045305169095);
#31303=CIRCLE('',#100410,60.4792282238308);
#31304=CIRCLE('',#100411,60.4792282238308);
#31305=CIRCLE('',#100412,60.4792282238308);
#31306=CIRCLE('',#100414,60.6419265158129);
#31307=CIRCLE('',#100416,60.8618969683742);
#31308=CIRCLE('',#100417,61.0131030316259);
#31309=CIRCLE('',#100419,61.2330734841871);
#31310=CIRCLE('',#100420,61.3957717761693);
#31311=CIRCLE('',#100421,61.3957717761693);
#31312=CIRCLE('',#100422,61.3957717761693);
#31313=CIRCLE('',#100424,61.8704694830905);
#31314=CIRCLE('',#100426,0.635007073208598);
#31315=CIRCLE('',#100427,0.63500707320861);
#31316=CIRCLE('',#100438,60.0045305169095);
#31317=CIRCLE('',#100439,60.4792282238308);
#31318=CIRCLE('',#100440,60.4792282238308);
#31319=CIRCLE('',#100441,60.4792282238308);
#31320=CIRCLE('',#100443,60.6419265158129);
#31321=CIRCLE('',#100445,60.8618969683742);
#31322=CIRCLE('',#100446,61.0131030316259);
#31323=CIRCLE('',#100448,61.2330734841871);
#31324=CIRCLE('',#100449,61.3957717761693);
#31325=CIRCLE('',#100450,61.3957717761693);
#31326=CIRCLE('',#100451,61.3957717761693);
#31327=CIRCLE('',#100453,61.8704694830905);
#31328=CIRCLE('',#100455,0.63500707320862);
#31329=CIRCLE('',#100456,0.635007073208583);
#31330=CIRCLE('',#100467,60.0045305169095);
#31331=CIRCLE('',#100468,60.4792282238308);
#31332=CIRCLE('',#100469,60.4792282238308);
#31333=CIRCLE('',#100470,60.4792282238308);
#31334=CIRCLE('',#100472,60.6419265158129);
#31335=CIRCLE('',#100474,60.8618969683742);
#31336=CIRCLE('',#100475,61.0131030316259);
#31337=CIRCLE('',#100477,61.2330734841871);
#31338=CIRCLE('',#100478,61.3957717761693);
#31339=CIRCLE('',#100479,61.3957717761693);
#31340=CIRCLE('',#100480,61.3957717761693);
#31341=CIRCLE('',#100482,61.8704694830905);
#31342=CIRCLE('',#100484,0.635007073208575);
#31343=CIRCLE('',#100485,0.635007073208584);
#31344=CIRCLE('',#100496,60.0045305169095);
#31345=CIRCLE('',#100497,60.4792282238308);
#31346=CIRCLE('',#100498,60.4792282238308);
#31347=CIRCLE('',#100499,60.4792282238308);
#31348=CIRCLE('',#100501,60.6419265158129);
#31349=CIRCLE('',#100503,60.8618969683742);
#31350=CIRCLE('',#100504,61.0131030316259);
#31351=CIRCLE('',#100506,61.2330734841871);
#31352=CIRCLE('',#100507,61.3957717761693);
#31353=CIRCLE('',#100508,61.3957717761693);
#31354=CIRCLE('',#100509,61.3957717761693);
#31355=CIRCLE('',#100511,61.8704694830905);
#31356=CIRCLE('',#100513,0.635007073208611);
#31357=CIRCLE('',#100514,0.635007073208621);
#31358=CIRCLE('',#100525,60.0045305169095);
#31359=CIRCLE('',#100526,60.4792282238308);
#31360=CIRCLE('',#100527,60.4792282238308);
#31361=CIRCLE('',#100528,60.4792282238308);
#31362=CIRCLE('',#100530,60.6419265158129);
#31363=CIRCLE('',#100532,60.8618969683742);
#31364=CIRCLE('',#100533,61.0131030316259);
#31365=CIRCLE('',#100535,61.2330734841871);
#31366=CIRCLE('',#100536,61.3957717761693);
#31367=CIRCLE('',#100537,61.3957717761693);
#31368=CIRCLE('',#100538,61.3957717761693);
#31369=CIRCLE('',#100540,61.8704694830905);
#31370=CIRCLE('',#100542,0.635007073208624);
#31371=CIRCLE('',#100543,0.63500707320863);
#31372=CIRCLE('',#100554,60.0045305169095);
#31373=CIRCLE('',#100555,60.4792282238308);
#31374=CIRCLE('',#100556,60.4792282238308);
#31375=CIRCLE('',#100557,60.4792282238308);
#31376=CIRCLE('',#100559,60.6419265158129);
#31377=CIRCLE('',#100561,60.8618969683742);
#31378=CIRCLE('',#100562,61.0131030316259);
#31379=CIRCLE('',#100564,61.2330734841871);
#31380=CIRCLE('',#100565,61.3957717761693);
#31381=CIRCLE('',#100566,61.3957717761693);
#31382=CIRCLE('',#100567,61.3957717761693);
#31383=CIRCLE('',#100569,61.8704694830905);
#31384=CIRCLE('',#100571,0.635007073208638);
#31385=CIRCLE('',#100572,0.635007073208613);
#31386=CIRCLE('',#100583,60.0045305169095);
#31387=CIRCLE('',#100584,60.4792282238308);
#31388=CIRCLE('',#100585,60.4792282238308);
#31389=CIRCLE('',#100586,60.4792282238308);
#31390=CIRCLE('',#100588,60.6419265158129);
#31391=CIRCLE('',#100590,60.8618969683742);
#31392=CIRCLE('',#100591,61.0131030316259);
#31393=CIRCLE('',#100593,61.2330734841871);
#31394=CIRCLE('',#100594,61.3957717761693);
#31395=CIRCLE('',#100595,61.3957717761693);
#31396=CIRCLE('',#100596,61.3957717761693);
#31397=CIRCLE('',#100598,61.8704694830905);
#31398=CIRCLE('',#100600,0.635007073208598);
#31399=CIRCLE('',#100601,0.635007073208607);
#31400=CIRCLE('',#100612,60.0045305169095);
#31401=CIRCLE('',#100613,60.4792282238308);
#31402=CIRCLE('',#100614,60.4792282238308);
#31403=CIRCLE('',#100615,60.4792282238308);
#31404=CIRCLE('',#100617,60.6419265158129);
#31405=CIRCLE('',#100619,60.8618969683742);
#31406=CIRCLE('',#100620,61.0131030316259);
#31407=CIRCLE('',#100622,61.2330734841871);
#31408=CIRCLE('',#100623,61.3957717761693);
#31409=CIRCLE('',#100624,61.3957717761693);
#31410=CIRCLE('',#100625,61.3957717761693);
#31411=CIRCLE('',#100627,61.8704694830905);
#31412=CIRCLE('',#100629,0.63500707320862);
#31413=CIRCLE('',#100630,0.635007073208593);
#31414=CIRCLE('',#100641,60.0045305169095);
#31415=CIRCLE('',#100642,60.4792282238308);
#31416=CIRCLE('',#100643,60.4792282238308);
#31417=CIRCLE('',#100644,60.4792282238308);
#31418=CIRCLE('',#100646,60.6419265158129);
#31419=CIRCLE('',#100648,60.8618969683742);
#31420=CIRCLE('',#100649,61.0131030316259);
#31421=CIRCLE('',#100651,61.2330734841871);
#31422=CIRCLE('',#100652,61.3957717761693);
#31423=CIRCLE('',#100653,61.3957717761693);
#31424=CIRCLE('',#100654,61.3957717761693);
#31425=CIRCLE('',#100656,61.8704694830905);
#31426=CIRCLE('',#100658,0.635007073208611);
#31427=CIRCLE('',#100659,0.635007073208634);
#31428=CIRCLE('',#100670,60.0045305169095);
#31429=CIRCLE('',#100671,60.4792282238308);
#31430=CIRCLE('',#100672,60.4792282238308);
#31431=CIRCLE('',#100673,60.4792282238308);
#31432=CIRCLE('',#100675,60.6419265158129);
#31433=CIRCLE('',#100677,60.8618969683742);
#31434=CIRCLE('',#100678,61.0131030316259);
#31435=CIRCLE('',#100680,61.2330734841871);
#31436=CIRCLE('',#100681,61.3957717761693);
#31437=CIRCLE('',#100682,61.3957717761693);
#31438=CIRCLE('',#100683,61.3957717761693);
#31439=CIRCLE('',#100685,61.8704694830905);
#31440=CIRCLE('',#100687,0.635007073208598);
#31441=CIRCLE('',#100688,0.635007073208591);
#31442=CIRCLE('',#100699,60.0045305169095);
#31443=CIRCLE('',#100700,60.4792282238308);
#31444=CIRCLE('',#100701,60.4792282238308);
#31445=CIRCLE('',#100702,60.4792282238308);
#31446=CIRCLE('',#100704,60.6419265158129);
#31447=CIRCLE('',#100706,60.8618969683742);
#31448=CIRCLE('',#100707,61.0131030316259);
#31449=CIRCLE('',#100709,61.2330734841871);
#31450=CIRCLE('',#100710,61.3957717761693);
#31451=CIRCLE('',#100711,61.3957717761693);
#31452=CIRCLE('',#100712,61.3957717761693);
#31453=CIRCLE('',#100714,61.8704694830905);
#31454=CIRCLE('',#100716,0.635007073208629);
#31455=CIRCLE('',#100717,0.635007073208631);
#31456=CIRCLE('',#100728,60.0045305169095);
#31457=CIRCLE('',#100729,60.4792282238308);
#31458=CIRCLE('',#100730,60.4792282238308);
#31459=CIRCLE('',#100731,60.4792282238308);
#31460=CIRCLE('',#100733,60.6419265158129);
#31461=CIRCLE('',#100735,60.8618969683742);
#31462=CIRCLE('',#100736,61.0131030316259);
#31463=CIRCLE('',#100738,61.2330734841871);
#31464=CIRCLE('',#100739,61.3957717761693);
#31465=CIRCLE('',#100740,61.3957717761693);
#31466=CIRCLE('',#100741,61.3957717761693);
#31467=CIRCLE('',#100743,61.8704694830905);
#31468=CIRCLE('',#100745,0.635007073208598);
#31469=CIRCLE('',#100746,0.635007073208607);
#31470=CIRCLE('',#100757,60.0045305169095);
#31471=CIRCLE('',#100758,60.4792282238308);
#31472=CIRCLE('',#100759,60.4792282238308);
#31473=CIRCLE('',#100760,60.4792282238308);
#31474=CIRCLE('',#100762,60.6419265158129);
#31475=CIRCLE('',#100764,60.8618969683742);
#31476=CIRCLE('',#100765,61.0131030316259);
#31477=CIRCLE('',#100767,61.2330734841871);
#31478=CIRCLE('',#100768,61.3957717761693);
#31479=CIRCLE('',#100769,61.3957717761693);
#31480=CIRCLE('',#100770,61.3957717761693);
#31481=CIRCLE('',#100772,61.8704694830905);
#31482=CIRCLE('',#100774,0.635007073208593);
#31483=CIRCLE('',#100775,0.63500707320864);
#31484=CIRCLE('',#100786,60.0045305169095);
#31485=CIRCLE('',#100787,60.4792282238308);
#31486=CIRCLE('',#100788,60.4792282238308);
#31487=CIRCLE('',#100789,60.4792282238308);
#31488=CIRCLE('',#100791,60.6419265158129);
#31489=CIRCLE('',#100793,60.8618969683742);
#31490=CIRCLE('',#100794,61.0131030316259);
#31491=CIRCLE('',#100796,61.2330734841871);
#31492=CIRCLE('',#100797,61.3957717761693);
#31493=CIRCLE('',#100798,61.3957717761693);
#31494=CIRCLE('',#100799,61.3957717761693);
#31495=CIRCLE('',#100801,61.8704694830905);
#31496=CIRCLE('',#100803,0.635007073208687);
#31497=CIRCLE('',#100804,0.635007073208632);
#31498=CIRCLE('',#100815,60.0045305169095);
#31499=CIRCLE('',#100816,60.4792282238308);
#31500=CIRCLE('',#100817,60.4792282238308);
#31501=CIRCLE('',#100818,60.4792282238308);
#31502=CIRCLE('',#100820,60.6419265158129);
#31503=CIRCLE('',#100822,60.8618969683742);
#31504=CIRCLE('',#100823,61.0131030316259);
#31505=CIRCLE('',#100825,61.2330734841871);
#31506=CIRCLE('',#100826,61.3957717761693);
#31507=CIRCLE('',#100827,61.3957717761693);
#31508=CIRCLE('',#100828,61.3957717761693);
#31509=CIRCLE('',#100830,61.8704694830905);
#31510=CIRCLE('',#100832,0.63500707320862);
#31511=CIRCLE('',#100833,0.635007073208634);
#31512=CIRCLE('',#100844,60.0045305169095);
#31513=CIRCLE('',#100845,60.4792282238308);
#31514=CIRCLE('',#100846,60.4792282238308);
#31515=CIRCLE('',#100847,60.4792282238308);
#31516=CIRCLE('',#100849,60.6419265158129);
#31517=CIRCLE('',#100851,60.8618969683742);
#31518=CIRCLE('',#100852,61.0131030316259);
#31519=CIRCLE('',#100854,61.2330734841871);
#31520=CIRCLE('',#100855,61.3957717761693);
#31521=CIRCLE('',#100856,61.3957717761693);
#31522=CIRCLE('',#100857,61.3957717761693);
#31523=CIRCLE('',#100859,61.8704694830905);
#31524=CIRCLE('',#100861,0.63500707320858);
#31525=CIRCLE('',#100862,0.635007073208591);
#31526=CIRCLE('',#100873,60.0045305169095);
#31527=CIRCLE('',#100874,60.4792282238308);
#31528=CIRCLE('',#100875,60.4792282238308);
#31529=CIRCLE('',#100876,60.4792282238308);
#31530=CIRCLE('',#100878,60.6419265158129);
#31531=CIRCLE('',#100880,60.8618969683742);
#31532=CIRCLE('',#100881,61.0131030316259);
#31533=CIRCLE('',#100883,61.2330734841871);
#31534=CIRCLE('',#100884,61.3957717761693);
#31535=CIRCLE('',#100885,61.3957717761693);
#31536=CIRCLE('',#100886,61.3957717761693);
#31537=CIRCLE('',#100888,61.8704694830905);
#31538=CIRCLE('',#100890,0.635007073208646);
#31539=CIRCLE('',#100891,0.635007073208626);
#31540=CIRCLE('',#100902,60.0045305169095);
#31541=CIRCLE('',#100903,60.4792282238308);
#31542=CIRCLE('',#100904,60.4792282238308);
#31543=CIRCLE('',#100905,60.4792282238308);
#31544=CIRCLE('',#100907,60.6419265158129);
#31545=CIRCLE('',#100909,60.8618969683742);
#31546=CIRCLE('',#100910,61.0131030316259);
#31547=CIRCLE('',#100912,61.2330734841871);
#31548=CIRCLE('',#100913,61.3957717761693);
#31549=CIRCLE('',#100914,61.3957717761693);
#31550=CIRCLE('',#100915,61.3957717761693);
#31551=CIRCLE('',#100917,61.8704694830905);
#31552=CIRCLE('',#100919,0.635007073208624);
#31553=CIRCLE('',#100920,0.635007073208612);
#31554=CIRCLE('',#100931,60.0045305169095);
#31555=CIRCLE('',#100932,60.4792282238308);
#31556=CIRCLE('',#100933,60.4792282238308);
#31557=CIRCLE('',#100934,60.4792282238308);
#31558=CIRCLE('',#100936,60.6419265158129);
#31559=CIRCLE('',#100938,60.8618969683742);
#31560=CIRCLE('',#100939,61.0131030316259);
#31561=CIRCLE('',#100941,61.2330734841871);
#31562=CIRCLE('',#100942,61.3957717761693);
#31563=CIRCLE('',#100943,61.3957717761693);
#31564=CIRCLE('',#100944,61.3957717761693);
#31565=CIRCLE('',#100946,61.8704694830905);
#31566=CIRCLE('',#100948,0.635007073208615);
#31567=CIRCLE('',#100949,0.63500707320861);
#31568=CIRCLE('',#100960,60.0045305169095);
#31569=CIRCLE('',#100961,60.4792282238308);
#31570=CIRCLE('',#100962,60.4792282238308);
#31571=CIRCLE('',#100963,60.4792282238308);
#31572=CIRCLE('',#100965,60.6419265158129);
#31573=CIRCLE('',#100967,60.8618969683742);
#31574=CIRCLE('',#100968,61.0131030316259);
#31575=CIRCLE('',#100970,61.2330734841871);
#31576=CIRCLE('',#100971,61.3957717761693);
#31577=CIRCLE('',#100972,61.3957717761693);
#31578=CIRCLE('',#100973,61.3957717761693);
#31579=CIRCLE('',#100975,61.8704694830905);
#31580=CIRCLE('',#100977,0.635007073208593);
#31581=CIRCLE('',#100978,0.635007073208623);
#31582=CIRCLE('',#100989,60.0045305169095);
#31583=CIRCLE('',#100990,60.4792282238308);
#31584=CIRCLE('',#100991,60.4792282238308);
#31585=CIRCLE('',#100992,60.4792282238308);
#31586=CIRCLE('',#100994,60.6419265158129);
#31587=CIRCLE('',#100996,60.8618969683742);
#31588=CIRCLE('',#100997,61.0131030316259);
#31589=CIRCLE('',#100999,61.2330734841871);
#31590=CIRCLE('',#101000,61.3957717761693);
#31591=CIRCLE('',#101001,61.3957717761693);
#31592=CIRCLE('',#101002,61.3957717761693);
#31593=CIRCLE('',#101004,61.8704694830905);
#31594=CIRCLE('',#101006,0.635007073208642);
#31595=CIRCLE('',#101007,0.635007073208646);
#31596=CIRCLE('',#101018,60.0045305169095);
#31597=CIRCLE('',#101019,60.4792282238308);
#31598=CIRCLE('',#101020,60.4792282238308);
#31599=CIRCLE('',#101021,60.4792282238308);
#31600=CIRCLE('',#101023,60.6419265158129);
#31601=CIRCLE('',#101025,60.8618969683742);
#31602=CIRCLE('',#101026,61.0131030316259);
#31603=CIRCLE('',#101028,61.2330734841871);
#31604=CIRCLE('',#101029,61.3957717761693);
#31605=CIRCLE('',#101030,61.3957717761693);
#31606=CIRCLE('',#101031,61.3957717761693);
#31607=CIRCLE('',#101033,61.8704694830905);
#31608=CIRCLE('',#101035,0.635007073208629);
#31609=CIRCLE('',#101036,0.635007073208629);
#31610=CIRCLE('',#101047,60.0045305169095);
#31611=CIRCLE('',#101048,60.4792282238308);
#31612=CIRCLE('',#101049,60.4792282238308);
#31613=CIRCLE('',#101050,60.4792282238308);
#31614=CIRCLE('',#101052,60.6419265158129);
#31615=CIRCLE('',#101054,60.8618969683742);
#31616=CIRCLE('',#101055,61.0131030316259);
#31617=CIRCLE('',#101057,61.2330734841871);
#31618=CIRCLE('',#101058,61.3957717761693);
#31619=CIRCLE('',#101059,61.3957717761693);
#31620=CIRCLE('',#101060,61.3957717761693);
#31621=CIRCLE('',#101062,61.8704694830905);
#31622=CIRCLE('',#101064,0.635007073208602);
#31623=CIRCLE('',#101065,0.635007073208621);
#31624=CIRCLE('',#101077,60.0045305169095);
#31625=CIRCLE('',#101078,60.4792282238308);
#31626=CIRCLE('',#101079,60.4792282238308);
#31627=CIRCLE('',#101080,60.4792282238308);
#31628=CIRCLE('',#101082,60.6419265158129);
#31629=CIRCLE('',#101084,60.8618969683742);
#31630=CIRCLE('',#101085,61.0131030316259);
#31631=CIRCLE('',#101087,61.2330734841871);
#31632=CIRCLE('',#101088,61.3957717761693);
#31633=CIRCLE('',#101089,61.3957717761693);
#31634=CIRCLE('',#101090,61.3957717761693);
#31635=CIRCLE('',#101092,61.8704694830905);
#31636=CIRCLE('',#101096,0.63500707320862);
#31637=CIRCLE('',#101097,0.635007073208634);
#31638=CIRCLE('',#101108,62.8464445485378);
#31639=CIRCLE('',#101109,59.0285554514622);
#31640=CIRCLE('',#101124,0.127);
#31641=CIRCLE('',#101125,0.127000000000002);
#31642=CIRCLE('',#101127,0.127000000000002);
#31643=CIRCLE('',#101129,0.127000000000002);
#31644=CIRCLE('',#101130,0.126999999999998);
#31645=CIRCLE('',#101131,0.127000000000001);
#31646=CIRCLE('',#101133,0.127000000000005);
#31647=CIRCLE('',#101136,0.127000000000002);
#31648=CIRCLE('',#101138,0.127000000000002);
#31649=CIRCLE('',#101140,0.127000000000002);
#31650=CIRCLE('',#101141,0.127000000000001);
#31651=CIRCLE('',#101142,0.127000000000005);
#31652=CIRCLE('',#101144,0.126999999999999);
#31653=CIRCLE('',#101146,0.126999999999998);
#31654=CIRCLE('',#101147,0.127000000000002);
#31655=CIRCLE('',#101148,0.127000000000002);
#31656=CIRCLE('',#101150,0.127000000000002);
#31657=CIRCLE('',#101153,0.126999999999999);
#31658=CIRCLE('',#101155,0.126999999999999);
#31659=CIRCLE('',#101157,0.127000000000001);
#31660=CIRCLE('',#101158,0.127000000000002);
#31661=CIRCLE('',#101159,0.127000000000002);
#31662=CIRCLE('',#101161,0.127000000000002);
#31663=CIRCLE('',#101164,0.127000000000001);
#31664=CIRCLE('',#101167,62.8464445485378);
#31665=CIRCLE('',#101168,59.0285554514622);
#31666=CIRCLE('',#101180,62.8464445485378);
#31667=CIRCLE('',#101181,59.0285554514622);
#31668=CIRCLE('',#101193,62.8464445485378);
#31669=CIRCLE('',#101194,59.0285554514622);
#31670=CIRCLE('',#101206,62.8464445485378);
#31671=CIRCLE('',#101207,59.0285554514622);
#31672=CIRCLE('',#101219,62.8464445485378);
#31673=CIRCLE('',#101220,59.0285554514622);
#31674=CIRCLE('',#101232,62.8464445485378);
#31675=CIRCLE('',#101233,59.0285554514622);
#31676=CIRCLE('',#101245,62.8464445485378);
#31677=CIRCLE('',#101246,59.0285554514622);
#31678=CIRCLE('',#101258,62.8464445485378);
#31679=CIRCLE('',#101259,59.0285554514622);
#31680=CIRCLE('',#101271,62.8464445485378);
#31681=CIRCLE('',#101272,59.0285554514622);
#31682=CIRCLE('',#101284,62.8464445485378);
#31683=CIRCLE('',#101285,59.0285554514622);
#31684=CIRCLE('',#101297,62.8464445485378);
#31685=CIRCLE('',#101298,59.0285554514622);
#31686=CIRCLE('',#101310,62.8464445485378);
#31687=CIRCLE('',#101311,59.0285554514622);
#31688=CIRCLE('',#101323,62.8464445485378);
#31689=CIRCLE('',#101324,59.0285554514622);
#31690=CIRCLE('',#101336,62.8464445485378);
#31691=CIRCLE('',#101337,59.0285554514622);
#31692=CIRCLE('',#101349,62.8464445485378);
#31693=CIRCLE('',#101350,59.0285554514622);
#31694=CIRCLE('',#101362,62.8464445485378);
#31695=CIRCLE('',#101363,59.0285554514622);
#31696=CIRCLE('',#101375,62.8464445485378);
#31697=CIRCLE('',#101376,59.0285554514622);
#31698=CIRCLE('',#101388,62.8464445485378);
#31699=CIRCLE('',#101389,59.0285554514622);
#31700=CIRCLE('',#101401,62.8464445485378);
#31701=CIRCLE('',#101402,59.0285554514622);
#31702=CIRCLE('',#101414,62.8464445485378);
#31703=CIRCLE('',#101415,59.0285554514622);
#31704=CIRCLE('',#101427,62.8464445485378);
#31705=CIRCLE('',#101428,59.0285554514622);
#31706=CIRCLE('',#101440,62.8464445485378);
#31707=CIRCLE('',#101441,59.0285554514622);
#31708=CIRCLE('',#101453,62.8464445485378);
#31709=CIRCLE('',#101454,59.0285554514622);
#31710=CIRCLE('',#101466,62.8464445485378);
#31711=CIRCLE('',#101467,59.0285554514622);
#31712=CIRCLE('',#101479,62.8464445485378);
#31713=CIRCLE('',#101480,59.0285554514622);
#31714=CIRCLE('',#101492,62.8464445485378);
#31715=CIRCLE('',#101493,59.0285554514622);
#31716=CIRCLE('',#101505,62.8464445485378);
#31717=CIRCLE('',#101506,59.0285554514622);
#31718=CIRCLE('',#101518,62.8464445485378);
#31719=CIRCLE('',#101519,59.0285554514622);
#31720=CIRCLE('',#101531,62.8464445485378);
#31721=CIRCLE('',#101532,59.0285554514622);
#31722=CIRCLE('',#101555,62.8464445485378);
#31723=CIRCLE('',#101556,59.0285554514622);
#31724=CIRCLE('',#101568,62.8464445485378);
#31725=CIRCLE('',#101569,59.0285554514622);
#31726=CIRCLE('',#101581,62.8464445485378);
#31727=CIRCLE('',#101582,59.0285554514622);
#31728=CIRCLE('',#101594,62.8464445485378);
#31729=CIRCLE('',#101595,59.0285554514622);
#31730=CIRCLE('',#101607,62.8464445485378);
#31731=CIRCLE('',#101608,59.0285554514622);
#31732=CIRCLE('',#101620,62.8464445485378);
#31733=CIRCLE('',#101621,59.0285554514622);
#31734=CIRCLE('',#101633,62.8464445485378);
#31735=CIRCLE('',#101634,59.0285554514622);
#31736=CIRCLE('',#101646,62.8464445485378);
#31737=CIRCLE('',#101647,59.0285554514622);
#31738=CIRCLE('',#101659,62.8464445485378);
#31739=CIRCLE('',#101660,59.0285554514622);
#31740=CIRCLE('',#101672,62.8464445485378);
#31741=CIRCLE('',#101673,59.0285554514622);
#31742=CIRCLE('',#101685,62.8464445485378);
#31743=CIRCLE('',#101686,59.0285554514622);
#31744=CIRCLE('',#101698,62.8464445485378);
#31745=CIRCLE('',#101699,59.0285554514622);
#31746=CIRCLE('',#101711,62.8464445485378);
#31747=CIRCLE('',#101712,59.0285554514622);
#31748=CIRCLE('',#101724,62.8464445485378);
#31749=CIRCLE('',#101725,59.0285554514622);
#31750=CIRCLE('',#101748,62.8464445485378);
#31751=CIRCLE('',#101749,59.0285554514622);
#31752=CIRCLE('',#101761,62.8464445485378);
#31753=CIRCLE('',#101762,59.0285554514622);
#31754=CIRCLE('',#101774,62.8464445485378);
#31755=CIRCLE('',#101775,59.0285554514622);
#31756=CIRCLE('',#101787,62.8464445485378);
#31757=CIRCLE('',#101788,59.0285554514622);
#31758=CIRCLE('',#101800,62.8464445485378);
#31759=CIRCLE('',#101801,59.0285554514622);
#31760=CIRCLE('',#101813,62.8464445485378);
#31761=CIRCLE('',#101814,59.0285554514622);
#31762=CIRCLE('',#101826,62.8464445485378);
#31763=CIRCLE('',#101827,59.0285554514622);
#31764=CIRCLE('',#101839,62.8464445485378);
#31765=CIRCLE('',#101840,59.0285554514622);
#31766=CIRCLE('',#101852,62.8464445485378);
#31767=CIRCLE('',#101853,59.0285554514622);
#31768=CIRCLE('',#101865,62.8464445485378);
#31769=CIRCLE('',#101866,59.0285554514622);
#31770=CIRCLE('',#101878,62.8464445485378);
#31771=CIRCLE('',#101879,59.0285554514622);
#31772=CIRCLE('',#101891,62.8464445485378);
#31773=CIRCLE('',#101892,59.0285554514622);
#31774=CIRCLE('',#101904,62.8464445485378);
#31775=CIRCLE('',#101905,59.0285554514622);
#31776=CIRCLE('',#101917,62.8464445485378);
#31777=CIRCLE('',#101918,59.0285554514622);
#31778=CIRCLE('',#102049,0.126999999999998);
#31779=CIRCLE('',#102050,0.127);
#31780=CIRCLE('',#102052,0.127);
#31781=CIRCLE('',#102054,0.127);
#31782=CIRCLE('',#102055,0.127);
#31783=CIRCLE('',#102056,0.127);
#31784=CIRCLE('',#102058,0.126999999999999);
#31785=CIRCLE('',#102061,0.127000000000004);
#31786=CIRCLE('',#102063,0.127);
#31787=CIRCLE('',#102065,0.127000000000002);
#31788=CIRCLE('',#102066,0.127000000000002);
#31789=CIRCLE('',#102067,0.126999999999997);
#31790=CIRCLE('',#102069,0.127000000000001);
#31791=CIRCLE('',#102071,0.127000000000004);
#31792=CIRCLE('',#102072,0.127);
#31793=CIRCLE('',#102073,0.127);
#31794=CIRCLE('',#102075,0.126999999999997);
#31795=CIRCLE('',#102078,0.127000000000001);
#31796=CIRCLE('',#102080,0.127000000000003);
#31797=CIRCLE('',#102082,0.127000000000004);
#31798=CIRCLE('',#102083,0.127);
#31799=CIRCLE('',#102084,0.127);
#31800=CIRCLE('',#102086,0.127);
#31801=CIRCLE('',#102089,0.127);
#31802=CIRCLE('',#102093,0.127000000000001);
#31803=CIRCLE('',#102094,0.126999999999999);
#31804=CIRCLE('',#102096,0.126999999999999);
#31805=CIRCLE('',#102098,0.126999999999999);
#31806=CIRCLE('',#102099,0.127000000000002);
#31807=CIRCLE('',#102100,0.127000000000003);
#31808=CIRCLE('',#102102,0.127000000000002);
#31809=CIRCLE('',#102105,0.127000000000003);
#31810=CIRCLE('',#102107,0.126999999999999);
#31811=CIRCLE('',#102109,0.126999999999997);
#31812=CIRCLE('',#102110,0.127);
#31813=CIRCLE('',#102111,0.127000000000002);
#31814=CIRCLE('',#102113,0.127000000000001);
#31815=CIRCLE('',#102115,0.126999999999999);
#31816=CIRCLE('',#102116,0.127000000000002);
#31817=CIRCLE('',#102117,0.126999999999999);
#31818=CIRCLE('',#102119,0.127000000000001);
#31819=CIRCLE('',#102122,0.127000000000001);
#31820=CIRCLE('',#102124,0.127000000000001);
#31821=CIRCLE('',#102126,0.127000000000002);
#31822=CIRCLE('',#102127,0.126999999999999);
#31823=CIRCLE('',#102128,0.126999999999999);
#31824=CIRCLE('',#102130,0.126999999999999);
#31825=CIRCLE('',#102133,0.127);
#31826=CIRCLE('',#102137,0.127000000000001);
#31827=CIRCLE('',#102138,0.126999999999999);
#31828=CIRCLE('',#102140,0.126999999999999);
#31829=CIRCLE('',#102142,0.127);
#31830=CIRCLE('',#102143,0.126999999999998);
#31831=CIRCLE('',#102144,0.126999999999997);
#31832=CIRCLE('',#102146,0.126999999999997);
#31833=CIRCLE('',#102149,0.126999999999997);
#31834=CIRCLE('',#102151,0.127);
#31835=CIRCLE('',#102153,0.127000000000001);
#31836=CIRCLE('',#102154,0.127000000000001);
#31837=CIRCLE('',#102155,0.127);
#31838=CIRCLE('',#102157,0.126999999999996);
#31839=CIRCLE('',#102159,0.127000000000002);
#31840=CIRCLE('',#102160,0.127000000000003);
#31841=CIRCLE('',#102161,0.126999999999999);
#31842=CIRCLE('',#102163,0.127);
#31843=CIRCLE('',#102166,0.126999999999996);
#31844=CIRCLE('',#102168,0.127000000000001);
#31845=CIRCLE('',#102170,0.127000000000001);
#31846=CIRCLE('',#102171,0.126999999999999);
#31847=CIRCLE('',#102172,0.126999999999999);
#31848=CIRCLE('',#102174,0.126999999999999);
#31849=CIRCLE('',#102177,0.127);
#31850=CIRCLE('',#102181,0.127);
#31851=CIRCLE('',#102182,0.127000000000001);
#31852=CIRCLE('',#102184,0.127000000000001);
#31853=CIRCLE('',#102186,0.127000000000001);
#31854=CIRCLE('',#102187,0.127000000000001);
#31855=CIRCLE('',#102188,0.127000000000001);
#31856=CIRCLE('',#102190,0.126999999999999);
#31857=CIRCLE('',#102193,0.127000000000002);
#31858=CIRCLE('',#102195,0.127000000000001);
#31859=CIRCLE('',#102197,0.127000000000001);
#31860=CIRCLE('',#102198,0.126999999999998);
#31861=CIRCLE('',#102199,0.126999999999999);
#31862=CIRCLE('',#102201,0.127);
#31863=CIRCLE('',#102203,0.127000000000004);
#31864=CIRCLE('',#102204,0.127000000000002);
#31865=CIRCLE('',#102205,0.127000000000001);
#31866=CIRCLE('',#102207,0.126999999999997);
#31867=CIRCLE('',#102210,0.127);
#31868=CIRCLE('',#102212,0.126999999999996);
#31869=CIRCLE('',#102214,0.126999999999998);
#31870=CIRCLE('',#102215,0.127000000000001);
#31871=CIRCLE('',#102216,0.127000000000001);
#31872=CIRCLE('',#102218,0.127000000000001);
#31873=CIRCLE('',#102221,0.127000000000001);
#31874=CIRCLE('',#102225,0.127000000000001);
#31875=CIRCLE('',#102226,0.127);
#31876=CIRCLE('',#102228,0.127);
#31877=CIRCLE('',#102230,0.127);
#31878=CIRCLE('',#102231,0.126999999999999);
#31879=CIRCLE('',#102232,0.126999999999998);
#31880=CIRCLE('',#102234,0.127);
#31881=CIRCLE('',#102237,0.127000000000002);
#31882=CIRCLE('',#102239,0.127);
#31883=CIRCLE('',#102241,0.127000000000002);
#31884=CIRCLE('',#102242,0.127000000000002);
#31885=CIRCLE('',#102243,0.127);
#31886=CIRCLE('',#102245,0.127000000000001);
#31887=CIRCLE('',#102247,0.126999999999999);
#31888=CIRCLE('',#102248,0.126999999999999);
#31889=CIRCLE('',#102249,0.127);
#31890=CIRCLE('',#102251,0.127000000000001);
#31891=CIRCLE('',#102254,0.127000000000001);
#31892=CIRCLE('',#102256,0.127000000000001);
#31893=CIRCLE('',#102258,0.126999999999999);
#31894=CIRCLE('',#102259,0.127);
#31895=CIRCLE('',#102260,0.127);
#31896=CIRCLE('',#102262,0.127);
#31897=CIRCLE('',#102265,0.126999999999998);
#31898=CIRCLE('',#102269,0.127000000000001);
#31899=CIRCLE('',#102270,0.126999999999999);
#31900=CIRCLE('',#102272,0.126999999999999);
#31901=CIRCLE('',#102274,0.127000000000004);
#31902=CIRCLE('',#102275,0.126999999999998);
#31903=CIRCLE('',#102276,0.126999999999997);
#31904=CIRCLE('',#102278,0.126999999999997);
#31905=CIRCLE('',#102281,0.126999999999999);
#31906=CIRCLE('',#102283,0.127);
#31907=CIRCLE('',#102285,0.127);
#31908=CIRCLE('',#102286,0.126999999999997);
#31909=CIRCLE('',#102287,0.126999999999997);
#31910=CIRCLE('',#102289,0.126999999999999);
#31911=CIRCLE('',#102291,0.126999999999998);
#31912=CIRCLE('',#102292,0.127000000000003);
#31913=CIRCLE('',#102293,0.126999999999999);
#31914=CIRCLE('',#102295,0.127);
#31915=CIRCLE('',#102298,0.127000000000003);
#31916=CIRCLE('',#102300,0.127000000000001);
#31917=CIRCLE('',#102302,0.127000000000004);
#31918=CIRCLE('',#102303,0.126999999999999);
#31919=CIRCLE('',#102304,0.127000000000004);
#31920=CIRCLE('',#102306,0.126999999999999);
#31921=CIRCLE('',#102309,0.126999999999997);
#31922=CIRCLE('',#102313,0.126999999999999);
#31923=CIRCLE('',#102314,0.127);
#31924=CIRCLE('',#102316,0.127);
#31925=CIRCLE('',#102318,0.127);
#31926=CIRCLE('',#102319,0.127000000000003);
#31927=CIRCLE('',#102320,0.127000000000001);
#31928=CIRCLE('',#102322,0.126999999999998);
#31929=CIRCLE('',#102325,0.127000000000003);
#31930=CIRCLE('',#102327,0.127);
#31931=CIRCLE('',#102329,0.126999999999999);
#31932=CIRCLE('',#102330,0.127000000000001);
#31933=CIRCLE('',#102331,0.126999999999998);
#31934=CIRCLE('',#102333,0.127000000000001);
#31935=CIRCLE('',#102335,0.126999999999997);
#31936=CIRCLE('',#102336,0.127000000000004);
#31937=CIRCLE('',#102337,0.127);
#31938=CIRCLE('',#102339,0.127000000000001);
#31939=CIRCLE('',#102342,0.126999999999998);
#31940=CIRCLE('',#102344,0.127000000000003);
#31941=CIRCLE('',#102346,0.127000000000001);
#31942=CIRCLE('',#102347,0.127);
#31943=CIRCLE('',#102348,0.127);
#31944=CIRCLE('',#102350,0.127);
#31945=CIRCLE('',#102353,0.127000000000001);
#31946=CIRCLE('',#102357,0.127000000000002);
#31947=CIRCLE('',#102358,0.127);
#31948=CIRCLE('',#102360,0.127);
#31949=CIRCLE('',#102362,0.127);
#31950=CIRCLE('',#102363,0.126999999999997);
#31951=CIRCLE('',#102364,0.127000000000001);
#31952=CIRCLE('',#102366,0.126999999999998);
#31953=CIRCLE('',#102369,0.126999999999999);
#31954=CIRCLE('',#102371,0.127);
#31955=CIRCLE('',#102373,0.127000000000003);
#31956=CIRCLE('',#102374,0.127000000000001);
#31957=CIRCLE('',#102375,0.126999999999998);
#31958=CIRCLE('',#102377,0.126999999999998);
#31959=CIRCLE('',#102379,0.126999999999997);
#31960=CIRCLE('',#102380,0.127000000000001);
#31961=CIRCLE('',#102381,0.127);
#31962=CIRCLE('',#102383,0.127);
#31963=CIRCLE('',#102386,0.127000000000001);
#31964=CIRCLE('',#102388,0.127000000000003);
#31965=CIRCLE('',#102390,0.126999999999998);
#31966=CIRCLE('',#102391,0.127);
#31967=CIRCLE('',#102392,0.127);
#31968=CIRCLE('',#102394,0.127);
#31969=CIRCLE('',#102397,0.127000000000001);
#31970=CIRCLE('',#102401,0.127000000000001);
#31971=CIRCLE('',#102402,0.127);
#31972=CIRCLE('',#102404,0.126999999999999);
#31973=CIRCLE('',#102406,0.127000000000004);
#31974=CIRCLE('',#102407,0.127000000000001);
#31975=CIRCLE('',#102408,0.127);
#31976=CIRCLE('',#102410,0.126999999999997);
#31977=CIRCLE('',#102413,0.126999999999995);
#31978=CIRCLE('',#102415,0.127);
#31979=CIRCLE('',#102417,0.126999999999998);
#31980=CIRCLE('',#102418,0.127000000000004);
#31981=CIRCLE('',#102419,0.126999999999997);
#31982=CIRCLE('',#102421,0.126999999999999);
#31983=CIRCLE('',#102423,0.127000000000001);
#31984=CIRCLE('',#102424,0.127000000000001);
#31985=CIRCLE('',#102425,0.126999999999999);
#31986=CIRCLE('',#102427,0.127000000000003);
#31987=CIRCLE('',#102430,0.126999999999999);
#31988=CIRCLE('',#102432,0.127000000000001);
#31989=CIRCLE('',#102434,0.127000000000004);
#31990=CIRCLE('',#102435,0.126999999999999);
#31991=CIRCLE('',#102436,0.126999999999999);
#31992=CIRCLE('',#102438,0.126999999999999);
#31993=CIRCLE('',#102441,0.126999999999997);
#31994=CIRCLE('',#102445,0.127000000000001);
#31995=CIRCLE('',#102446,0.127);
#31996=CIRCLE('',#102448,0.127);
#31997=CIRCLE('',#102450,0.127);
#31998=CIRCLE('',#102451,0.126999999999999);
#31999=CIRCLE('',#102452,0.126999999999998);
#32000=CIRCLE('',#102454,0.127);
#32001=CIRCLE('',#102457,0.127000000000002);
#32002=CIRCLE('',#102459,0.127);
#32003=CIRCLE('',#102461,0.126999999999999);
#32004=CIRCLE('',#102462,0.126999999999996);
#32005=CIRCLE('',#102463,0.127);
#32006=CIRCLE('',#102465,0.127000000000001);
#32007=CIRCLE('',#102467,0.126999999999999);
#32008=CIRCLE('',#102468,0.127);
#32009=CIRCLE('',#102469,0.127);
#32010=CIRCLE('',#102471,0.126999999999999);
#32011=CIRCLE('',#102474,0.127000000000001);
#32012=CIRCLE('',#102476,0.127000000000001);
#32013=CIRCLE('',#102478,0.126999999999996);
#32014=CIRCLE('',#102479,0.127);
#32015=CIRCLE('',#102480,0.127);
#32016=CIRCLE('',#102482,0.127);
#32017=CIRCLE('',#102485,0.126999999999998);
#32018=CIRCLE('',#102489,0.126999999999997);
#32019=CIRCLE('',#102490,0.127000000000001);
#32020=CIRCLE('',#102492,0.127000000000001);
#32021=CIRCLE('',#102494,0.127000000000001);
#32022=CIRCLE('',#102495,0.127000000000001);
#32023=CIRCLE('',#102496,0.127000000000001);
#32024=CIRCLE('',#102498,0.126999999999996);
#32025=CIRCLE('',#102501,0.127000000000001);
#32026=CIRCLE('',#102503,0.127000000000001);
#32027=CIRCLE('',#102505,0.127000000000001);
#32028=CIRCLE('',#102506,0.126999999999998);
#32029=CIRCLE('',#102507,0.126999999999999);
#32030=CIRCLE('',#102509,0.127);
#32031=CIRCLE('',#102511,0.127000000000001);
#32032=CIRCLE('',#102512,0.126999999999997);
#32033=CIRCLE('',#102513,0.127000000000001);
#32034=CIRCLE('',#102515,0.127000000000001);
#32035=CIRCLE('',#102518,0.126999999999997);
#32036=CIRCLE('',#102520,0.127);
#32037=CIRCLE('',#102522,0.126999999999998);
#32038=CIRCLE('',#102523,0.127000000000001);
#32039=CIRCLE('',#102524,0.127000000000001);
#32040=CIRCLE('',#102526,0.127000000000001);
#32041=CIRCLE('',#102529,0.127000000000004);
#32042=CIRCLE('',#102533,0.126999999999999);
#32043=CIRCLE('',#102534,0.127000000000002);
#32044=CIRCLE('',#102536,0.126999999999999);
#32045=CIRCLE('',#102538,0.126999999999999);
#32046=CIRCLE('',#102539,0.127000000000002);
#32047=CIRCLE('',#102540,0.127);
#32048=CIRCLE('',#102542,0.126999999999997);
#32049=CIRCLE('',#102545,0.127);
#32050=CIRCLE('',#102547,0.127);
#32051=CIRCLE('',#102549,0.126999999999998);
#32052=CIRCLE('',#102550,0.127000000000001);
#32053=CIRCLE('',#102551,0.126999999999997);
#32054=CIRCLE('',#102553,0.126999999999996);
#32055=CIRCLE('',#102555,0.126999999999998);
#32056=CIRCLE('',#102556,0.127);
#32057=CIRCLE('',#102557,0.126999999999999);
#32058=CIRCLE('',#102559,0.127000000000003);
#32059=CIRCLE('',#102562,0.126999999999996);
#32060=CIRCLE('',#102564,0.127000000000001);
#32061=CIRCLE('',#102566,0.127000000000001);
#32062=CIRCLE('',#102567,0.126999999999999);
#32063=CIRCLE('',#102568,0.126999999999999);
#32064=CIRCLE('',#102570,0.126999999999999);
#32065=CIRCLE('',#102573,0.127);
#32066=CIRCLE('',#102577,0.127000000000001);
#32067=CIRCLE('',#102578,0.126999999999999);
#32068=CIRCLE('',#102580,0.126999999999999);
#32069=CIRCLE('',#102582,0.126999999999999);
#32070=CIRCLE('',#102583,0.127000000000002);
#32071=CIRCLE('',#102584,0.127000000000003);
#32072=CIRCLE('',#102586,0.127000000000002);
#32073=CIRCLE('',#102589,0.126999999999997);
#32074=CIRCLE('',#102591,0.126999999999999);
#32075=CIRCLE('',#102593,0.126999999999996);
#32076=CIRCLE('',#102594,0.127000000000002);
#32077=CIRCLE('',#102595,0.127);
#32078=CIRCLE('',#102597,0.127000000000001);
#32079=CIRCLE('',#102599,0.127000000000002);
#32080=CIRCLE('',#102600,0.127);
#32081=CIRCLE('',#102601,0.126999999999999);
#32082=CIRCLE('',#102603,0.127000000000002);
#32083=CIRCLE('',#102606,0.127000000000001);
#32084=CIRCLE('',#102608,0.126999999999998);
#32085=CIRCLE('',#102610,0.126999999999996);
#32086=CIRCLE('',#102611,0.126999999999999);
#32087=CIRCLE('',#102612,0.126999999999999);
#32088=CIRCLE('',#102614,0.126999999999999);
#32089=CIRCLE('',#102617,0.127);
#32090=CIRCLE('',#102621,0.127000000000004);
#32091=CIRCLE('',#102622,0.127);
#32092=CIRCLE('',#102624,0.127);
#32093=CIRCLE('',#102626,0.127);
#32094=CIRCLE('',#102627,0.127);
#32095=CIRCLE('',#102628,0.127);
#32096=CIRCLE('',#102630,0.126999999999999);
#32097=CIRCLE('',#102633,0.127000000000002);
#32098=CIRCLE('',#102635,0.127);
#32099=CIRCLE('',#102637,0.127000000000004);
#32100=CIRCLE('',#102638,0.126999999999998);
#32101=CIRCLE('',#102639,0.126999999999999);
#32102=CIRCLE('',#102641,0.127000000000001);
#32103=CIRCLE('',#102643,0.126999999999998);
#32104=CIRCLE('',#102644,0.126999999999997);
#32105=CIRCLE('',#102645,0.127);
#32106=CIRCLE('',#102647,0.127);
#32107=CIRCLE('',#102650,0.127000000000001);
#32108=CIRCLE('',#102652,0.127000000000003);
#32109=CIRCLE('',#102654,0.126999999999998);
#32110=CIRCLE('',#102655,0.127);
#32111=CIRCLE('',#102656,0.127);
#32112=CIRCLE('',#102658,0.127);
#32113=CIRCLE('',#102661,0.127);
#32114=CIRCLE('',#102665,0.127);
#32115=CIRCLE('',#102666,0.127000000000002);
#32116=CIRCLE('',#102668,0.127000000000002);
#32117=CIRCLE('',#102670,0.127000000000002);
#32118=CIRCLE('',#102671,0.126999999999998);
#32119=CIRCLE('',#102672,0.127000000000001);
#32120=CIRCLE('',#102674,0.127000000000005);
#32121=CIRCLE('',#102677,0.127000000000002);
#32122=CIRCLE('',#102679,0.127000000000002);
#32123=CIRCLE('',#102681,0.127000000000002);
#32124=CIRCLE('',#102682,0.127000000000001);
#32125=CIRCLE('',#102683,0.126999999999997);
#32126=CIRCLE('',#102685,0.126999999999999);
#32127=CIRCLE('',#102687,0.126999999999998);
#32128=CIRCLE('',#102688,0.127000000000002);
#32129=CIRCLE('',#102689,0.127000000000002);
#32130=CIRCLE('',#102691,0.127000000000002);
#32131=CIRCLE('',#102694,0.126999999999999);
#32132=CIRCLE('',#102696,0.127000000000003);
#32133=CIRCLE('',#102698,0.127000000000001);
#32134=CIRCLE('',#102699,0.127000000000002);
#32135=CIRCLE('',#102700,0.127000000000002);
#32136=CIRCLE('',#102702,0.127000000000002);
#32137=CIRCLE('',#102705,0.127000000000001);
#32138=CIRCLE('',#102709,0.126999999999998);
#32139=CIRCLE('',#102710,0.127);
#32140=CIRCLE('',#102712,0.127);
#32141=CIRCLE('',#102714,0.127);
#32142=CIRCLE('',#102715,0.126999999999998);
#32143=CIRCLE('',#102716,0.127);
#32144=CIRCLE('',#102718,0.126999999999999);
#32145=CIRCLE('',#102721,0.127000000000004);
#32146=CIRCLE('',#102723,0.127);
#32147=CIRCLE('',#102725,0.127000000000002);
#32148=CIRCLE('',#102726,0.126999999999998);
#32149=CIRCLE('',#102727,0.126999999999999);
#32150=CIRCLE('',#102729,0.127000000000001);
#32151=CIRCLE('',#102731,0.127000000000004);
#32152=CIRCLE('',#102732,0.127);
#32153=CIRCLE('',#102733,0.127);
#32154=CIRCLE('',#102735,0.126999999999997);
#32155=CIRCLE('',#102738,0.127000000000001);
#32156=CIRCLE('',#102740,0.127000000000003);
#32157=CIRCLE('',#102742,0.127000000000004);
#32158=CIRCLE('',#102743,0.127);
#32159=CIRCLE('',#102744,0.127);
#32160=CIRCLE('',#102746,0.127);
#32161=CIRCLE('',#102749,0.127);
#32162=CIRCLE('',#102753,0.127000000000001);
#32163=CIRCLE('',#102754,0.126999999999999);
#32164=CIRCLE('',#102756,0.126999999999999);
#32165=CIRCLE('',#102758,0.126999999999999);
#32166=CIRCLE('',#102759,0.126999999999999);
#32167=CIRCLE('',#102760,0.127);
#32168=CIRCLE('',#102762,0.127000000000002);
#32169=CIRCLE('',#102765,0.126999999999997);
#32170=CIRCLE('',#102767,0.126999999999999);
#32171=CIRCLE('',#102769,0.126999999999997);
#32172=CIRCLE('',#102770,0.127);
#32173=CIRCLE('',#102771,0.127000000000002);
#32174=CIRCLE('',#102773,0.127000000000001);
#32175=CIRCLE('',#102775,0.126999999999999);
#32176=CIRCLE('',#102776,0.127000000000002);
#32177=CIRCLE('',#102777,0.126999999999999);
#32178=CIRCLE('',#102779,0.127000000000001);
#32179=CIRCLE('',#102782,0.127000000000001);
#32180=CIRCLE('',#102784,0.126999999999997);
#32181=CIRCLE('',#102786,0.127000000000002);
#32182=CIRCLE('',#102787,0.126999999999999);
#32183=CIRCLE('',#102788,0.126999999999999);
#32184=CIRCLE('',#102790,0.126999999999999);
#32185=CIRCLE('',#102793,0.127);
#32186=CIRCLE('',#102797,0.127000000000001);
#32187=CIRCLE('',#102798,0.126999999999999);
#32188=CIRCLE('',#102800,0.126999999999999);
#32189=CIRCLE('',#102802,0.127);
#32190=CIRCLE('',#102803,0.126999999999998);
#32191=CIRCLE('',#102804,0.127);
#32192=CIRCLE('',#102806,0.126999999999997);
#32193=CIRCLE('',#102809,0.126999999999998);
#32194=CIRCLE('',#102811,0.126999999999999);
#32195=CIRCLE('',#102813,0.127);
#32196=CIRCLE('',#102814,0.127000000000001);
#32197=CIRCLE('',#102815,0.127000000000003);
#32198=CIRCLE('',#102817,0.126999999999996);
#32199=CIRCLE('',#102819,0.127000000000002);
#32200=CIRCLE('',#102820,0.126999999999997);
#32201=CIRCLE('',#102821,0.126999999999999);
#32202=CIRCLE('',#102823,0.127);
#32203=CIRCLE('',#102826,0.126999999999999);
#32204=CIRCLE('',#102828,0.127000000000004);
#32205=CIRCLE('',#102830,0.127000000000001);
#32206=CIRCLE('',#102831,0.126999999999999);
#32207=CIRCLE('',#102832,0.126999999999999);
#32208=CIRCLE('',#102834,0.126999999999999);
#32209=CIRCLE('',#102837,0.127);
#32210=CIRCLE('',#102841,0.127);
#32211=CIRCLE('',#102842,0.127000000000001);
#32212=CIRCLE('',#102844,0.127000000000001);
#32213=CIRCLE('',#102846,0.127000000000001);
#32214=CIRCLE('',#102847,0.127000000000001);
#32215=CIRCLE('',#102848,0.127000000000001);
#32216=CIRCLE('',#102850,0.126999999999999);
#32217=CIRCLE('',#102853,0.127000000000002);
#32218=CIRCLE('',#102855,0.127000000000001);
#32219=CIRCLE('',#102857,0.127000000000001);
#32220=CIRCLE('',#102858,0.126999999999998);
#32221=CIRCLE('',#102859,0.126999999999996);
#32222=CIRCLE('',#102861,0.127);
#32223=CIRCLE('',#102863,0.127000000000001);
#32224=CIRCLE('',#102864,0.127000000000002);
#32225=CIRCLE('',#102865,0.127000000000001);
#32226=CIRCLE('',#102867,0.126999999999998);
#32227=CIRCLE('',#102870,0.127);
#32228=CIRCLE('',#102872,0.127);
#32229=CIRCLE('',#102874,0.127000000000004);
#32230=CIRCLE('',#102875,0.127000000000001);
#32231=CIRCLE('',#102876,0.127000000000001);
#32232=CIRCLE('',#102878,0.127000000000001);
#32233=CIRCLE('',#102881,0.126999999999998);
#32234=CIRCLE('',#102885,0.127000000000001);
#32235=CIRCLE('',#102886,0.127);
#32236=CIRCLE('',#102888,0.127000000000003);
#32237=CIRCLE('',#102890,0.127);
#32238=CIRCLE('',#102891,0.127000000000002);
#32239=CIRCLE('',#102892,0.127000000000001);
#32240=CIRCLE('',#102894,0.127);
#32241=CIRCLE('',#102897,0.126999999999998);
#32242=CIRCLE('',#102899,0.127);
#32243=CIRCLE('',#102901,0.127000000000002);
#32244=CIRCLE('',#102902,0.127000000000002);
#32245=CIRCLE('',#102903,0.127);
#32246=CIRCLE('',#102905,0.127000000000001);
#32247=CIRCLE('',#102907,0.127000000000002);
#32248=CIRCLE('',#102908,0.126999999999999);
#32249=CIRCLE('',#102909,0.127);
#32250=CIRCLE('',#102911,0.127);
#32251=CIRCLE('',#102914,0.127000000000001);
#32252=CIRCLE('',#102916,0.127000000000001);
#32253=CIRCLE('',#102918,0.127000000000002);
#32254=CIRCLE('',#102919,0.127);
#32255=CIRCLE('',#102920,0.127);
#32256=CIRCLE('',#102922,0.127);
#32257=CIRCLE('',#102925,0.126999999999998);
#32258=CIRCLE('',#102929,0.127000000000001);
#32259=CIRCLE('',#102930,0.127000000000004);
#32260=CIRCLE('',#102932,0.126999999999999);
#32261=CIRCLE('',#102934,0.127000000000004);
#32262=CIRCLE('',#102935,0.126999999999998);
#32263=CIRCLE('',#102936,0.126999999999997);
#32264=CIRCLE('',#102938,0.127);
#32265=CIRCLE('',#102941,0.126999999999998);
#32266=CIRCLE('',#102943,0.127000000000004);
#32267=CIRCLE('',#102945,0.126999999999995);
#32268=CIRCLE('',#102946,0.126999999999997);
#32269=CIRCLE('',#102947,0.127);
#32270=CIRCLE('',#102949,0.126999999999999);
#32271=CIRCLE('',#102951,0.126999999999998);
#32272=CIRCLE('',#102952,0.127000000000003);
#32273=CIRCLE('',#102953,0.126999999999999);
#32274=CIRCLE('',#102955,0.127);
#32275=CIRCLE('',#102958,0.127000000000002);
#32276=CIRCLE('',#102960,0.126999999999998);
#32277=CIRCLE('',#102962,0.127);
#32278=CIRCLE('',#102963,0.126999999999999);
#32279=CIRCLE('',#102964,0.126999999999999);
#32280=CIRCLE('',#102966,0.126999999999999);
#32281=CIRCLE('',#102969,0.126999999999997);
#32282=CIRCLE('',#102973,0.126999999999999);
#32283=CIRCLE('',#102974,0.127);
#32284=CIRCLE('',#102976,0.127);
#32285=CIRCLE('',#102978,0.127);
#32286=CIRCLE('',#102979,0.126999999999997);
#32287=CIRCLE('',#102980,0.127000000000001);
#32288=CIRCLE('',#102982,0.126999999999998);
#32289=CIRCLE('',#102985,0.126999999999998);
#32290=CIRCLE('',#102987,0.127);
#32291=CIRCLE('',#102989,0.126999999999998);
#32292=CIRCLE('',#102990,0.127000000000001);
#32293=CIRCLE('',#102991,0.126999999999998);
#32294=CIRCLE('',#102993,0.127000000000001);
#32295=CIRCLE('',#102995,0.127000000000003);
#32296=CIRCLE('',#102996,0.127);
#32297=CIRCLE('',#102997,0.127);
#32298=CIRCLE('',#102999,0.126999999999996);
#32299=CIRCLE('',#103002,0.126999999999998);
#32300=CIRCLE('',#103004,0.126999999999999);
#32301=CIRCLE('',#103006,0.127000000000001);
#32302=CIRCLE('',#103007,0.127);
#32303=CIRCLE('',#103008,0.127);
#32304=CIRCLE('',#103010,0.127);
#32305=CIRCLE('',#103013,0.127000000000001);
#32306=CIRCLE('',#103017,0.126999999999999);
#32307=CIRCLE('',#103018,0.127);
#32308=CIRCLE('',#103020,0.127);
#32309=CIRCLE('',#103022,0.127);
#32310=CIRCLE('',#103023,0.127000000000003);
#32311=CIRCLE('',#103024,0.127000000000001);
#32312=CIRCLE('',#103026,0.127000000000002);
#32313=CIRCLE('',#103029,0.126999999999999);
#32314=CIRCLE('',#103031,0.127);
#32315=CIRCLE('',#103033,0.127000000000003);
#32316=CIRCLE('',#103034,0.127000000000004);
#32317=CIRCLE('',#103035,0.127000000000001);
#32318=CIRCLE('',#103037,0.126999999999998);
#32319=CIRCLE('',#103039,0.126999999999997);
#32320=CIRCLE('',#103040,0.127000000000001);
#32321=CIRCLE('',#103041,0.127);
#32322=CIRCLE('',#103043,0.127);
#32323=CIRCLE('',#103046,0.127000000000001);
#32324=CIRCLE('',#103048,0.126999999999999);
#32325=CIRCLE('',#103050,0.127000000000001);
#32326=CIRCLE('',#103051,0.127);
#32327=CIRCLE('',#103052,0.127);
#32328=CIRCLE('',#103054,0.127);
#32329=CIRCLE('',#103057,0.127000000000001);
#32330=CIRCLE('',#103061,0.127000000000001);
#32331=CIRCLE('',#103062,0.127000000000004);
#32332=CIRCLE('',#103064,0.127000000000004);
#32333=CIRCLE('',#103066,0.127);
#32334=CIRCLE('',#103067,0.127000000000001);
#32335=CIRCLE('',#103068,0.126999999999997);
#32336=CIRCLE('',#103070,0.127);
#32337=CIRCLE('',#103073,0.126999999999995);
#32338=CIRCLE('',#103075,0.127000000000004);
#32339=CIRCLE('',#103077,0.126999999999998);
#32340=CIRCLE('',#103078,0.127000000000001);
#32341=CIRCLE('',#103079,0.127);
#32342=CIRCLE('',#103081,0.126999999999999);
#32343=CIRCLE('',#103083,0.127000000000001);
#32344=CIRCLE('',#103084,0.127);
#32345=CIRCLE('',#103085,0.127000000000004);
#32346=CIRCLE('',#103087,0.127000000000003);
#32347=CIRCLE('',#103090,0.126999999999999);
#32348=CIRCLE('',#103092,0.127000000000001);
#32349=CIRCLE('',#103094,0.127000000000004);
#32350=CIRCLE('',#103095,0.127000000000004);
#32351=CIRCLE('',#103096,0.127);
#32352=CIRCLE('',#103098,0.127000000000004);
#32353=CIRCLE('',#103101,0.127);
#32354=CIRCLE('',#103105,0.127000000000001);
#32355=CIRCLE('',#103106,0.127);
#32356=CIRCLE('',#103108,0.127);
#32357=CIRCLE('',#103110,0.127);
#32358=CIRCLE('',#103111,0.126999999999999);
#32359=CIRCLE('',#103112,0.127000000000001);
#32360=CIRCLE('',#103114,0.127);
#32361=CIRCLE('',#103117,0.127000000000002);
#32362=CIRCLE('',#103119,0.126999999999999);
#32363=CIRCLE('',#103121,0.127000000000002);
#32364=CIRCLE('',#103122,0.127000000000002);
#32365=CIRCLE('',#103123,0.127);
#32366=CIRCLE('',#103125,0.126999999999998);
#32367=CIRCLE('',#103127,0.126999999999999);
#32368=CIRCLE('',#103128,0.127);
#32369=CIRCLE('',#103129,0.127000000000003);
#32370=CIRCLE('',#103131,0.126999999999998);
#32371=CIRCLE('',#103134,0.127000000000001);
#32372=CIRCLE('',#103136,0.126999999999998);
#32373=CIRCLE('',#103138,0.127000000000002);
#32374=CIRCLE('',#103139,0.127);
#32375=CIRCLE('',#103140,0.127);
#32376=CIRCLE('',#103142,0.127);
#32377=CIRCLE('',#103145,0.126999999999998);
#32378=CIRCLE('',#103149,0.127);
#32379=CIRCLE('',#103150,0.127000000000001);
#32380=CIRCLE('',#103152,0.127000000000001);
#32381=CIRCLE('',#103154,0.127000000000001);
#32382=CIRCLE('',#103155,0.127000000000001);
#32383=CIRCLE('',#103156,0.127000000000004);
#32384=CIRCLE('',#103158,0.126999999999999);
#32385=CIRCLE('',#103161,0.127000000000002);
#32386=CIRCLE('',#103163,0.127000000000001);
#32387=CIRCLE('',#103165,0.127000000000001);
#32388=CIRCLE('',#103166,0.127000000000001);
#32389=CIRCLE('',#103167,0.126999999999999);
#32390=CIRCLE('',#103169,0.126999999999997);
#32391=CIRCLE('',#103171,0.126999999999997);
#32392=CIRCLE('',#103172,0.127000000000003);
#32393=CIRCLE('',#103173,0.127000000000001);
#32394=CIRCLE('',#103175,0.127000000000001);
#32395=CIRCLE('',#103178,0.127);
#32396=CIRCLE('',#103180,0.127);
#32397=CIRCLE('',#103182,0.126999999999998);
#32398=CIRCLE('',#103183,0.127000000000001);
#32399=CIRCLE('',#103184,0.127000000000001);
#32400=CIRCLE('',#103186,0.127000000000001);
#32401=CIRCLE('',#103189,0.127000000000001);
#32402=CIRCLE('',#103193,0.126999999999999);
#32403=CIRCLE('',#103194,0.126999999999999);
#32404=CIRCLE('',#103196,0.126999999999999);
#32405=CIRCLE('',#103198,0.126999999999999);
#32406=CIRCLE('',#103199,0.126999999999998);
#32407=CIRCLE('',#103200,0.127);
#32408=CIRCLE('',#103202,0.126999999999997);
#32409=CIRCLE('',#103205,0.127);
#32410=CIRCLE('',#103207,0.127);
#32411=CIRCLE('',#103209,0.126999999999998);
#32412=CIRCLE('',#103210,0.127000000000001);
#32413=CIRCLE('',#103211,0.126999999999997);
#32414=CIRCLE('',#103213,0.126999999999996);
#32415=CIRCLE('',#103215,0.127000000000002);
#32416=CIRCLE('',#103216,0.126999999999999);
#32417=CIRCLE('',#103217,0.126999999999999);
#32418=CIRCLE('',#103219,0.127000000000002);
#32419=CIRCLE('',#103222,0.126999999999996);
#32420=CIRCLE('',#103224,0.127000000000001);
#32421=CIRCLE('',#103226,0.127000000000001);
#32422=CIRCLE('',#103227,0.126999999999999);
#32423=CIRCLE('',#103228,0.127);
#32424=CIRCLE('',#103230,0.126999999999999);
#32425=CIRCLE('',#103233,0.127000000000003);
#32426=CIRCLE('',#103237,0.127000000000001);
#32427=CIRCLE('',#103238,0.127000000000001);
#32428=CIRCLE('',#103240,0.126999999999999);
#32429=CIRCLE('',#103242,0.127000000000001);
#32430=CIRCLE('',#103243,0.127000000000002);
#32431=CIRCLE('',#103244,0.127);
#32432=CIRCLE('',#103246,0.127000000000002);
#32433=CIRCLE('',#103249,0.126999999999997);
#32434=CIRCLE('',#103251,0.126999999999999);
#32435=CIRCLE('',#103253,0.126999999999997);
#32436=CIRCLE('',#103254,0.127);
#32437=CIRCLE('',#103255,0.126999999999999);
#32438=CIRCLE('',#103257,0.127000000000001);
#32439=CIRCLE('',#103259,0.126999999999999);
#32440=CIRCLE('',#103260,0.127);
#32441=CIRCLE('',#103261,0.126999999999999);
#32442=CIRCLE('',#103263,0.127000000000002);
#32443=CIRCLE('',#103266,0.127000000000001);
#32444=CIRCLE('',#103268,0.127000000000001);
#32445=CIRCLE('',#103270,0.126999999999996);
#32446=CIRCLE('',#103271,0.126999999999999);
#32447=CIRCLE('',#103272,0.126999999999999);
#32448=CIRCLE('',#103274,0.126999999999999);
#32449=CIRCLE('',#103277,0.127);
#32450=CIRCLE('',#103281,0.127000000000004);
#32451=CIRCLE('',#103282,0.127);
#32452=CIRCLE('',#103284,0.127);
#32453=CIRCLE('',#103286,0.127);
#32454=CIRCLE('',#103287,0.126999999999998);
#32455=CIRCLE('',#103288,0.127);
#32456=CIRCLE('',#103290,0.126999999999999);
#32457=CIRCLE('',#103293,0.127000000000002);
#32458=CIRCLE('',#103295,0.127);
#32459=CIRCLE('',#103297,0.127000000000004);
#32460=CIRCLE('',#103298,0.127000000000004);
#32461=CIRCLE('',#103299,0.126999999999999);
#32462=CIRCLE('',#103301,0.127000000000001);
#32463=CIRCLE('',#103303,0.126999999999998);
#32464=CIRCLE('',#103304,0.126999999999997);
#32465=CIRCLE('',#103305,0.127);
#32466=CIRCLE('',#103307,0.127);
#32467=CIRCLE('',#103310,0.127000000000001);
#32468=CIRCLE('',#103312,0.127000000000003);
#32469=CIRCLE('',#103314,0.126999999999998);
#32470=CIRCLE('',#103315,0.127);
#32471=CIRCLE('',#103316,0.127);
#32472=CIRCLE('',#103318,0.127);
#32473=CIRCLE('',#103321,0.127);
#32474=CIRCLE('',#103325,0.127);
#32475=CIRCLE('',#103326,0.127000000000002);
#32476=CIRCLE('',#103328,0.127000000000002);
#32477=CIRCLE('',#103330,0.127000000000002);
#32478=CIRCLE('',#103331,0.126999999999998);
#32479=CIRCLE('',#103332,0.127000000000001);
#32480=CIRCLE('',#103334,0.127000000000005);
#32481=CIRCLE('',#103338,0.127000000000002);
#32482=CIRCLE('',#103339,0.127000000000001);
#32483=CIRCLE('',#103340,0.127000000000005);
#32484=CIRCLE('',#103342,0.126999999999999);
#32485=CIRCLE('',#103344,0.126999999999998);
#32486=CIRCLE('',#103345,0.127000000000002);
#32487=CIRCLE('',#103348,0.126999999999999);
#32488=CIRCLE('',#103350,0.126999999999999);
#32489=CIRCLE('',#103352,0.127000000000001);
#32490=CIRCLE('',#103353,0.127000000000002);
#32491=CIRCLE('',#103354,0.127000000000002);
#32492=CIRCLE('',#103356,0.127000000000002);
#32493=CIRCLE('',#103359,0.127000000000001);
#32494=CIRCLE('',#103363,0.126999999999998);
#32495=CIRCLE('',#103364,0.127);
#32496=CIRCLE('',#103366,0.127);
#32497=CIRCLE('',#103368,0.127);
#32498=CIRCLE('',#103369,0.126999999999998);
#32499=CIRCLE('',#103370,0.127);
#32500=CIRCLE('',#103372,0.126999999999999);
#32501=CIRCLE('',#103375,0.127000000000004);
#32502=CIRCLE('',#103377,0.127);
#32503=CIRCLE('',#103379,0.127000000000002);
#32504=CIRCLE('',#103380,0.126999999999998);
#32505=CIRCLE('',#103381,0.126999999999999);
#32506=CIRCLE('',#103383,0.127000000000001);
#32507=CIRCLE('',#103385,0.126999999999996);
#32508=CIRCLE('',#103386,0.127);
#32509=CIRCLE('',#103387,0.127);
#32510=CIRCLE('',#103389,0.126999999999997);
#32511=CIRCLE('',#103392,0.127000000000001);
#32512=CIRCLE('',#103394,0.127000000000003);
#32513=CIRCLE('',#103396,0.127000000000004);
#32514=CIRCLE('',#103397,0.127);
#32515=CIRCLE('',#103398,0.127);
#32516=CIRCLE('',#103400,0.127);
#32517=CIRCLE('',#103403,0.127);
#32518=CIRCLE('',#103407,0.127000000000001);
#32519=CIRCLE('',#103408,0.126999999999999);
#32520=CIRCLE('',#103410,0.126999999999999);
#32521=CIRCLE('',#103412,0.126999999999999);
#32522=CIRCLE('',#103413,0.127000000000002);
#32523=CIRCLE('',#103414,0.127);
#32524=CIRCLE('',#103416,0.127000000000002);
#32525=CIRCLE('',#103419,0.126999999999997);
#32526=CIRCLE('',#103421,0.126999999999999);
#32527=CIRCLE('',#103423,0.126999999999997);
#32528=CIRCLE('',#103424,0.126999999999996);
#32529=CIRCLE('',#103425,0.127000000000002);
#32530=CIRCLE('',#103427,0.127000000000001);
#32531=CIRCLE('',#103429,0.127000000000002);
#32532=CIRCLE('',#103430,0.127000000000002);
#32533=CIRCLE('',#103431,0.126999999999999);
#32534=CIRCLE('',#103433,0.127000000000001);
#32535=CIRCLE('',#103436,0.127000000000001);
#32536=CIRCLE('',#103438,0.127000000000001);
#32537=CIRCLE('',#103440,0.127000000000002);
#32538=CIRCLE('',#103441,0.126999999999999);
#32539=CIRCLE('',#103442,0.126999999999999);
#32540=CIRCLE('',#103444,0.126999999999999);
#32541=CIRCLE('',#103447,0.127000000000003);
#32542=CIRCLE('',#103451,0.127000000000001);
#32543=CIRCLE('',#103452,0.126999999999999);
#32544=CIRCLE('',#103454,0.126999999999999);
#32545=CIRCLE('',#103456,0.127000000000002);
#32546=CIRCLE('',#103457,0.126999999999998);
#32547=CIRCLE('',#103458,0.127);
#32548=CIRCLE('',#103460,0.126999999999997);
#32549=CIRCLE('',#103463,0.126999999999999);
#32550=CIRCLE('',#103465,0.127000000000002);
#32551=CIRCLE('',#103467,0.127000000000001);
#32552=CIRCLE('',#103468,0.127000000000001);
#32553=CIRCLE('',#103469,0.127);
#32554=CIRCLE('',#103471,0.126999999999999);
#32555=CIRCLE('',#103473,0.126999999999998);
#32556=CIRCLE('',#103474,0.126999999999997);
#32557=CIRCLE('',#103475,0.126999999999999);
#32558=CIRCLE('',#103477,0.127);
#32559=CIRCLE('',#103480,0.127000000000002);
#32560=CIRCLE('',#103482,0.127000000000001);
#32561=CIRCLE('',#103484,0.126999999999997);
#32562=CIRCLE('',#103485,0.126999999999999);
#32563=CIRCLE('',#103486,0.126999999999999);
#32564=CIRCLE('',#103488,0.126999999999999);
#32565=CIRCLE('',#103491,0.127);
#32566=CIRCLE('',#103495,0.127);
#32567=CIRCLE('',#103496,0.127000000000001);
#32568=CIRCLE('',#103498,0.127000000000001);
#32569=CIRCLE('',#103500,0.127000000000001);
#32570=CIRCLE('',#103501,0.127000000000001);
#32571=CIRCLE('',#103502,0.127000000000004);
#32572=CIRCLE('',#103504,0.126999999999999);
#32573=CIRCLE('',#103507,0.127000000000002);
#32574=CIRCLE('',#103509,0.127000000000001);
#32575=CIRCLE('',#103511,0.127000000000001);
#32576=CIRCLE('',#103512,0.127000000000001);
#32577=CIRCLE('',#103513,0.127000000000002);
#32578=CIRCLE('',#103515,0.127);
#32579=CIRCLE('',#103517,0.127000000000001);
#32580=CIRCLE('',#103518,0.127000000000002);
#32581=CIRCLE('',#103519,0.127000000000001);
#32582=CIRCLE('',#103521,0.126999999999998);
#32583=CIRCLE('',#103524,0.126999999999997);
#32584=CIRCLE('',#103526,0.127);
#32585=CIRCLE('',#103528,0.127000000000004);
#32586=CIRCLE('',#103529,0.127000000000001);
#32587=CIRCLE('',#103530,0.127000000000001);
#32588=CIRCLE('',#103532,0.127000000000001);
#32589=CIRCLE('',#103535,0.127000000000001);
#32590=CIRCLE('',#103539,0.127000000000001);
#32591=CIRCLE('',#103540,0.127);
#32592=CIRCLE('',#103542,0.127);
#32593=CIRCLE('',#103544,0.127);
#32594=CIRCLE('',#103545,0.126999999999999);
#32595=CIRCLE('',#103546,0.126999999999998);
#32596=CIRCLE('',#103548,0.127);
#32597=CIRCLE('',#103551,0.127000000000002);
#32598=CIRCLE('',#103553,0.127);
#32599=CIRCLE('',#103555,0.127000000000002);
#32600=CIRCLE('',#103556,0.126999999999999);
#32601=CIRCLE('',#103557,0.127);
#32602=CIRCLE('',#103559,0.127000000000001);
#32603=CIRCLE('',#103561,0.126999999999999);
#32604=CIRCLE('',#103562,0.126999999999999);
#32605=CIRCLE('',#103563,0.127);
#32606=CIRCLE('',#103565,0.127000000000001);
#32607=CIRCLE('',#103568,0.127000000000001);
#32608=CIRCLE('',#103570,0.127000000000001);
#32609=CIRCLE('',#103572,0.126999999999999);
#32610=CIRCLE('',#103573,0.127);
#32611=CIRCLE('',#103574,0.127);
#32612=CIRCLE('',#103576,0.127);
#32613=CIRCLE('',#103579,0.126999999999998);
#32614=CIRCLE('',#103583,0.127000000000001);
#32615=CIRCLE('',#103584,0.127000000000004);
#32616=CIRCLE('',#103586,0.126999999999999);
#32617=CIRCLE('',#103588,0.127000000000004);
#32618=CIRCLE('',#103589,0.126999999999998);
#32619=CIRCLE('',#103590,0.126999999999997);
#32620=CIRCLE('',#103592,0.127);
#32621=CIRCLE('',#103595,0.126999999999998);
#32622=CIRCLE('',#103597,0.127000000000003);
#32623=CIRCLE('',#103599,0.126999999999995);
#32624=CIRCLE('',#103600,0.127000000000001);
#32625=CIRCLE('',#103601,0.127);
#32626=CIRCLE('',#103603,0.126999999999999);
#32627=CIRCLE('',#103605,0.127000000000001);
#32628=CIRCLE('',#103606,0.127000000000003);
#32629=CIRCLE('',#103607,0.126999999999999);
#32630=CIRCLE('',#103609,0.127);
#32631=CIRCLE('',#103612,0.126999999999999);
#32632=CIRCLE('',#103614,0.127000000000001);
#32633=CIRCLE('',#103616,0.126999999999997);
#32634=CIRCLE('',#103617,0.126999999999999);
#32635=CIRCLE('',#103618,0.126999999999999);
#32636=CIRCLE('',#103620,0.126999999999999);
#32637=CIRCLE('',#103623,0.126999999999997);
#32638=CIRCLE('',#103627,0.126999999999999);
#32639=CIRCLE('',#103628,0.127);
#32640=CIRCLE('',#103630,0.127);
#32641=CIRCLE('',#103632,0.127);
#32642=CIRCLE('',#103633,0.126999999999997);
#32643=CIRCLE('',#103634,0.127000000000001);
#32644=CIRCLE('',#103636,0.127000000000002);
#32645=CIRCLE('',#103639,0.127000000000003);
#32646=CIRCLE('',#103641,0.127);
#32647=CIRCLE('',#103643,0.126999999999998);
#32648=CIRCLE('',#103644,0.127000000000001);
#32649=CIRCLE('',#103645,0.126999999999998);
#32650=CIRCLE('',#103647,0.127000000000001);
#32651=CIRCLE('',#103649,0.127000000000003);
#32652=CIRCLE('',#103650,0.127);
#32653=CIRCLE('',#103651,0.127);
#32654=CIRCLE('',#103653,0.126999999999996);
#32655=CIRCLE('',#103656,0.126999999999998);
#32656=CIRCLE('',#103658,0.126999999999997);
#32657=CIRCLE('',#103660,0.127000000000001);
#32658=CIRCLE('',#103661,0.127);
#32659=CIRCLE('',#103662,0.127);
#32660=CIRCLE('',#103664,0.127);
#32661=CIRCLE('',#103667,0.127000000000001);
#32662=CIRCLE('',#103671,0.126999999999999);
#32663=CIRCLE('',#103672,0.127);
#32664=CIRCLE('',#103674,0.127);
#32665=CIRCLE('',#103676,0.127);
#32666=CIRCLE('',#103677,0.127000000000003);
#32667=CIRCLE('',#103678,0.126999999999998);
#32668=CIRCLE('',#103680,0.126999999999998);
#32669=CIRCLE('',#103683,0.126999999999999);
#32670=CIRCLE('',#103685,0.127);
#32671=CIRCLE('',#103687,0.127000000000003);
#32672=CIRCLE('',#103688,0.126999999999998);
#32673=CIRCLE('',#103689,0.126999999999998);
#32674=CIRCLE('',#103691,0.126999999999998);
#32675=CIRCLE('',#103693,0.126999999999997);
#32676=CIRCLE('',#103694,0.127000000000001);
#32677=CIRCLE('',#103695,0.127);
#32678=CIRCLE('',#103697,0.127);
#32679=CIRCLE('',#103700,0.127000000000001);
#32680=CIRCLE('',#103702,0.127000000000003);
#32681=CIRCLE('',#103704,0.126999999999998);
#32682=CIRCLE('',#103705,0.127);
#32683=CIRCLE('',#103706,0.127);
#32684=CIRCLE('',#103708,0.127);
#32685=CIRCLE('',#103711,0.127000000000004);
#32686=CIRCLE('',#103715,0.127000000000001);
#32687=CIRCLE('',#103716,0.127000000000004);
#32688=CIRCLE('',#103718,0.127000000000004);
#32689=CIRCLE('',#103720,0.127000000000004);
#32690=CIRCLE('',#103721,0.127000000000001);
#32691=CIRCLE('',#103722,0.127);
#32692=CIRCLE('',#103724,0.127);
#32693=CIRCLE('',#103727,0.126999999999995);
#32694=CIRCLE('',#103729,0.127000000000004);
#32695=CIRCLE('',#103731,0.126999999999998);
#32696=CIRCLE('',#103732,0.127);
#32697=CIRCLE('',#103733,0.126999999999997);
#32698=CIRCLE('',#103735,0.126999999999999);
#32699=CIRCLE('',#103737,0.127000000000001);
#32700=CIRCLE('',#103738,0.127);
#32701=CIRCLE('',#103739,0.127000000000004);
#32702=CIRCLE('',#103741,0.127000000000003);
#32703=CIRCLE('',#103744,0.127000000000003);
#32704=CIRCLE('',#103746,0.126999999999998);
#32705=CIRCLE('',#103748,0.126999999999997);
#32706=CIRCLE('',#103749,0.127000000000004);
#32707=CIRCLE('',#103750,0.126999999999999);
#32708=CIRCLE('',#103752,0.127000000000004);
#32709=CIRCLE('',#103755,0.126999999999997);
#32710=CIRCLE('',#103759,0.127000000000001);
#32711=CIRCLE('',#103760,0.127);
#32712=CIRCLE('',#103762,0.127);
#32713=CIRCLE('',#103764,0.127);
#32714=CIRCLE('',#103765,0.126999999999999);
#32715=CIRCLE('',#103766,0.127000000000001);
#32716=CIRCLE('',#103768,0.127);
#32717=CIRCLE('',#103771,0.127000000000002);
#32718=CIRCLE('',#103773,0.127);
#32719=CIRCLE('',#103775,0.127000000000002);
#32720=CIRCLE('',#103776,0.127000000000002);
#32721=CIRCLE('',#103777,0.127);
#32722=CIRCLE('',#103779,0.127000000000001);
#32723=CIRCLE('',#103781,0.127000000000002);
#32724=CIRCLE('',#103782,0.127);
#32725=CIRCLE('',#103783,0.127000000000003);
#32726=CIRCLE('',#103785,0.126999999999999);
#32727=CIRCLE('',#103788,0.127000000000001);
#32728=CIRCLE('',#103790,0.126999999999998);
#32729=CIRCLE('',#103792,0.127000000000002);
#32730=CIRCLE('',#103793,0.127);
#32731=CIRCLE('',#103794,0.127);
#32732=CIRCLE('',#103796,0.127);
#32733=CIRCLE('',#103799,0.127000000000001);
#32734=CIRCLE('',#103803,0.127);
#32735=CIRCLE('',#103804,0.127000000000001);
#32736=CIRCLE('',#103806,0.127000000000001);
#32737=CIRCLE('',#103808,0.127000000000001);
#32738=CIRCLE('',#103809,0.127000000000004);
#32739=CIRCLE('',#103810,0.127000000000004);
#32740=CIRCLE('',#103812,0.126999999999999);
#32741=CIRCLE('',#103815,0.126999999999999);
#32742=CIRCLE('',#103817,0.127000000000001);
#32743=CIRCLE('',#103819,0.127000000000002);
#32744=CIRCLE('',#103820,0.127000000000001);
#32745=CIRCLE('',#103821,0.126999999999999);
#32746=CIRCLE('',#103823,0.127);
#32747=CIRCLE('',#103825,0.127000000000001);
#32748=CIRCLE('',#103826,0.127000000000003);
#32749=CIRCLE('',#103827,0.127000000000001);
#32750=CIRCLE('',#103829,0.127000000000001);
#32751=CIRCLE('',#103832,0.127);
#32752=CIRCLE('',#103834,0.127000000000003);
#32753=CIRCLE('',#103836,0.126999999999998);
#32754=CIRCLE('',#103837,0.127000000000001);
#32755=CIRCLE('',#103838,0.127000000000001);
#32756=CIRCLE('',#103840,0.127000000000001);
#32757=CIRCLE('',#103843,0.127000000000001);
#32758=CIRCLE('',#103847,0.126999999999999);
#32759=CIRCLE('',#103848,0.127);
#32760=CIRCLE('',#103850,0.127);
#32761=CIRCLE('',#103852,0.126999999999999);
#32762=CIRCLE('',#103853,0.126999999999998);
#32763=CIRCLE('',#103854,0.127);
#32764=CIRCLE('',#103856,0.127);
#32765=CIRCLE('',#103859,0.127);
#32766=CIRCLE('',#103861,0.127);
#32767=CIRCLE('',#103863,0.126999999999998);
#32768=CIRCLE('',#103864,0.127000000000001);
#32769=CIRCLE('',#103865,0.126999999999997);
#32770=CIRCLE('',#103867,0.126999999999999);
#32771=CIRCLE('',#103869,0.127000000000002);
#32772=CIRCLE('',#103870,0.126999999999999);
#32773=CIRCLE('',#103871,0.127);
#32774=CIRCLE('',#103873,0.127000000000002);
#32775=CIRCLE('',#103876,0.126999999999999);
#32776=CIRCLE('',#103878,0.127000000000001);
#32777=CIRCLE('',#103880,0.127000000000001);
#32778=CIRCLE('',#103881,0.127);
#32779=CIRCLE('',#103882,0.127);
#32780=CIRCLE('',#103884,0.127);
#32781=CIRCLE('',#103887,0.127);
#32782=CIRCLE('',#103891,0.127000000000001);
#32783=CIRCLE('',#103892,0.126999999999999);
#32784=CIRCLE('',#103894,0.126999999999999);
#32785=CIRCLE('',#103896,0.126999999999999);
#32786=CIRCLE('',#103897,0.127000000000002);
#32787=CIRCLE('',#103898,0.127);
#32788=CIRCLE('',#103900,0.126999999999996);
#32789=CIRCLE('',#103903,0.127000000000003);
#32790=CIRCLE('',#103905,0.126999999999999);
#32791=CIRCLE('',#103907,0.127000000000003);
#32792=CIRCLE('',#103908,0.127);
#32793=CIRCLE('',#103909,0.127000000000002);
#32794=CIRCLE('',#103911,0.127000000000001);
#32795=CIRCLE('',#103913,0.127000000000002);
#32796=CIRCLE('',#103914,0.127);
#32797=CIRCLE('',#103915,0.126999999999999);
#32798=CIRCLE('',#103917,0.127000000000002);
#32799=CIRCLE('',#103920,0.126999999999999);
#32800=CIRCLE('',#103922,0.127000000000001);
#32801=CIRCLE('',#103924,0.127);
#32802=CIRCLE('',#103925,0.126999999999999);
#32803=CIRCLE('',#103926,0.126999999999999);
#32804=CIRCLE('',#103928,0.126999999999999);
#32805=CIRCLE('',#103931,0.127);
#32806=CIRCLE('',#103935,0.126999999999998);
#32807=CIRCLE('',#103936,0.127);
#32808=CIRCLE('',#103938,0.127);
#32809=CIRCLE('',#103940,0.127);
#32810=CIRCLE('',#103941,0.126999999999998);
#32811=CIRCLE('',#103942,0.127);
#32812=CIRCLE('',#103944,0.126999999999999);
#32813=CIRCLE('',#103947,0.127000000000002);
#32814=CIRCLE('',#103949,0.127);
#32815=CIRCLE('',#103951,0.127000000000004);
#32816=CIRCLE('',#103952,0.126999999999998);
#32817=CIRCLE('',#103953,0.126999999999999);
#32818=CIRCLE('',#103955,0.127000000000001);
#32819=CIRCLE('',#103957,0.127);
#32820=CIRCLE('',#103958,0.126999999999997);
#32821=CIRCLE('',#103959,0.127);
#32822=CIRCLE('',#103961,0.127);
#32823=CIRCLE('',#103964,0.127000000000001);
#32824=CIRCLE('',#103966,0.127000000000003);
#32825=CIRCLE('',#103968,0.126999999999998);
#32826=CIRCLE('',#103969,0.127);
#32827=CIRCLE('',#103970,0.127);
#32828=CIRCLE('',#103972,0.127);
#32829=CIRCLE('',#103975,0.126999999999997);
#32830=CIRCLE('',#103979,0.127);
#32831=CIRCLE('',#103980,0.127000000000002);
#32832=CIRCLE('',#103982,0.127000000000002);
#32833=CIRCLE('',#103984,0.127000000000002);
#32834=CIRCLE('',#103985,0.126999999999998);
#32835=CIRCLE('',#103986,0.127000000000001);
#32836=CIRCLE('',#103988,0.127000000000005);
#32837=CIRCLE('',#103992,0.127000000000002);
#32838=CIRCLE('',#103993,0.127000000000001);
#32839=CIRCLE('',#103994,0.127000000000005);
#32840=CIRCLE('',#103996,0.126999999999999);
#32841=CIRCLE('',#103998,0.126999999999998);
#32842=CIRCLE('',#103999,0.127000000000002);
#32843=CIRCLE('',#104002,0.126999999999999);
#32844=CIRCLE('',#104004,0.126999999999997);
#32845=CIRCLE('',#104006,0.127000000000001);
#32846=CIRCLE('',#104007,0.127000000000002);
#32847=CIRCLE('',#104008,0.127000000000002);
#32848=CIRCLE('',#104010,0.127000000000002);
#32849=CIRCLE('',#104013,0.127000000000001);
#32850=CIRCLE('',#104017,0.126999999999998);
#32851=CIRCLE('',#104018,0.127);
#32852=CIRCLE('',#104020,0.127);
#32853=CIRCLE('',#104022,0.127);
#32854=CIRCLE('',#104023,0.126999999999998);
#32855=CIRCLE('',#104024,0.127);
#32856=CIRCLE('',#104026,0.126999999999999);
#32857=CIRCLE('',#104029,0.127000000000004);
#32858=CIRCLE('',#104031,0.127);
#32859=CIRCLE('',#104033,0.127000000000002);
#32860=CIRCLE('',#104034,0.126999999999998);
#32861=CIRCLE('',#104035,0.126999999999999);
#32862=CIRCLE('',#104037,0.127000000000001);
#32863=CIRCLE('',#104039,0.127000000000004);
#32864=CIRCLE('',#104040,0.127);
#32865=CIRCLE('',#104041,0.127);
#32866=CIRCLE('',#104043,0.126999999999997);
#32867=CIRCLE('',#104046,0.127000000000001);
#32868=CIRCLE('',#104048,0.127000000000003);
#32869=CIRCLE('',#104050,0.127000000000004);
#32870=CIRCLE('',#104051,0.127);
#32871=CIRCLE('',#104052,0.127);
#32872=CIRCLE('',#104054,0.127);
#32873=CIRCLE('',#104057,0.126999999999997);
#32874=CIRCLE('',#104061,0.127000000000001);
#32875=CIRCLE('',#104062,0.126999999999999);
#32876=CIRCLE('',#104064,0.126999999999999);
#32877=CIRCLE('',#104066,0.126999999999999);
#32878=CIRCLE('',#104067,0.127000000000002);
#32879=CIRCLE('',#104068,0.127);
#32880=CIRCLE('',#104070,0.126999999999999);
#32881=CIRCLE('',#104073,0.126999999999997);
#32882=CIRCLE('',#104075,0.127000000000001);
#32883=CIRCLE('',#104077,0.126999999999997);
#32884=CIRCLE('',#104078,0.126999999999996);
#32885=CIRCLE('',#104079,0.126999999999999);
#32886=CIRCLE('',#104081,0.127000000000001);
#32887=CIRCLE('',#104083,0.127000000000002);
#32888=CIRCLE('',#104084,0.127000000000002);
#32889=CIRCLE('',#104085,0.126999999999999);
#32890=CIRCLE('',#104087,0.127000000000001);
#32891=CIRCLE('',#104090,0.127000000000001);
#32892=CIRCLE('',#104092,0.127000000000001);
#32893=CIRCLE('',#104094,0.126999999999996);
#32894=CIRCLE('',#104095,0.126999999999999);
#32895=CIRCLE('',#104096,0.126999999999999);
#32896=CIRCLE('',#104098,0.126999999999999);
#32897=CIRCLE('',#104101,0.127);
#32898=CIRCLE('',#104105,0.127000000000001);
#32899=CIRCLE('',#104106,0.126999999999999);
#32900=CIRCLE('',#104108,0.126999999999999);
#32901=CIRCLE('',#104110,0.127);
#32902=CIRCLE('',#104111,0.126999999999998);
#32903=CIRCLE('',#104112,0.126999999999997);
#32904=CIRCLE('',#104114,0.127000000000003);
#32905=CIRCLE('',#104117,0.126999999999998);
#32906=CIRCLE('',#104119,0.126999999999999);
#32907=CIRCLE('',#104121,0.127000000000001);
#32908=CIRCLE('',#104122,0.127000000000001);
#32909=CIRCLE('',#104123,0.126999999999999);
#32910=CIRCLE('',#104125,0.127000000000002);
#32911=CIRCLE('',#104127,0.126999999999998);
#32912=CIRCLE('',#104128,0.126999999999997);
#32913=CIRCLE('',#104129,0.126999999999999);
#32914=CIRCLE('',#104131,0.127);
#32915=CIRCLE('',#104134,0.126999999999999);
#32916=CIRCLE('',#104136,0.126999999999998);
#32917=CIRCLE('',#104138,0.127000000000001);
#32918=CIRCLE('',#104139,0.126999999999999);
#32919=CIRCLE('',#104140,0.126999999999999);
#32920=CIRCLE('',#104142,0.126999999999999);
#32921=CIRCLE('',#104145,0.127);
#32922=CIRCLE('',#104149,0.127);
#32923=CIRCLE('',#104150,0.127000000000001);
#32924=CIRCLE('',#104152,0.127000000000001);
#32925=CIRCLE('',#104154,0.127000000000001);
#32926=CIRCLE('',#104155,0.127000000000001);
#32927=CIRCLE('',#104156,0.127000000000004);
#32928=CIRCLE('',#104158,0.126999999999996);
#32929=CIRCLE('',#104161,0.127000000000002);
#32930=CIRCLE('',#104163,0.127000000000001);
#32931=CIRCLE('',#104165,0.127000000000001);
#32932=CIRCLE('',#104166,0.126999999999998);
#32933=CIRCLE('',#104167,0.126999999999999);
#32934=CIRCLE('',#104169,0.126999999999997);
#32935=CIRCLE('',#104171,0.127000000000001);
#32936=CIRCLE('',#104172,0.127000000000001);
#32937=CIRCLE('',#104173,0.127000000000001);
#32938=CIRCLE('',#104175,0.126999999999998);
#32939=CIRCLE('',#104178,0.127);
#32940=CIRCLE('',#104180,0.127000000000003);
#32941=CIRCLE('',#104182,0.127000000000004);
#32942=CIRCLE('',#104183,0.127000000000001);
#32943=CIRCLE('',#104184,0.127000000000001);
#32944=CIRCLE('',#104186,0.127000000000001);
#32945=CIRCLE('',#104189,0.127000000000001);
#32946=CIRCLE('',#104193,0.127000000000001);
#32947=CIRCLE('',#104194,0.127);
#32948=CIRCLE('',#104196,0.127000000000003);
#32949=CIRCLE('',#104198,0.127);
#32950=CIRCLE('',#104199,0.126999999999999);
#32951=CIRCLE('',#104200,0.126999999999998);
#32952=CIRCLE('',#104202,0.127);
#32953=CIRCLE('',#104205,0.126999999999998);
#32954=CIRCLE('',#104207,0.127);
#32955=CIRCLE('',#104209,0.126999999999996);
#32956=CIRCLE('',#104210,0.127000000000002);
#32957=CIRCLE('',#104211,0.126999999999996);
#32958=CIRCLE('',#104213,0.127000000000001);
#32959=CIRCLE('',#104215,0.127000000000002);
#32960=CIRCLE('',#104216,0.126999999999999);
#32961=CIRCLE('',#104217,0.127);
#32962=CIRCLE('',#104219,0.127000000000001);
#32963=CIRCLE('',#104222,0.126999999999998);
#32964=CIRCLE('',#104224,0.127000000000001);
#32965=CIRCLE('',#104226,0.126999999999999);
#32966=CIRCLE('',#104227,0.127);
#32967=CIRCLE('',#104228,0.127);
#32968=CIRCLE('',#104230,0.127);
#32969=CIRCLE('',#104233,0.126999999999998);
#32970=CIRCLE('',#104237,0.127000000000004);
#32971=CIRCLE('',#104238,0.126999999999999);
#32972=CIRCLE('',#104240,0.126999999999999);
#32973=CIRCLE('',#104242,0.127000000000004);
#32974=CIRCLE('',#104243,0.126999999999998);
#32975=CIRCLE('',#104244,0.126999999999997);
#32976=CIRCLE('',#104246,0.127);
#32977=CIRCLE('',#104249,0.126999999999998);
#32978=CIRCLE('',#104251,0.127000000000004);
#32979=CIRCLE('',#104253,0.127);
#32980=CIRCLE('',#104254,0.126999999999997);
#32981=CIRCLE('',#104255,0.126999999999997);
#32982=CIRCLE('',#104257,0.127000000000003);
#32983=CIRCLE('',#104259,0.126999999999998);
#32984=CIRCLE('',#104260,0.127000000000003);
#32985=CIRCLE('',#104261,0.126999999999999);
#32986=CIRCLE('',#104263,0.127);
#32987=CIRCLE('',#104266,0.126999999999999);
#32988=CIRCLE('',#104268,0.127000000000004);
#32989=CIRCLE('',#104270,0.127);
#32990=CIRCLE('',#104271,0.126999999999999);
#32991=CIRCLE('',#104272,0.126999999999999);
#32992=CIRCLE('',#104274,0.126999999999999);
#32993=CIRCLE('',#104277,0.126999999999997);
#32994=CIRCLE('',#104281,0.126999999999999);
#32995=CIRCLE('',#104282,0.127);
#32996=CIRCLE('',#104284,0.127);
#32997=CIRCLE('',#104286,0.127);
#32998=CIRCLE('',#104287,0.127000000000003);
#32999=CIRCLE('',#104288,0.127000000000001);
#33000=CIRCLE('',#104290,0.126999999999998);
#33001=CIRCLE('',#104293,0.126999999999998);
#33002=CIRCLE('',#104295,0.127);
#33003=CIRCLE('',#104297,0.126999999999998);
#33004=CIRCLE('',#104298,0.127000000000001);
#33005=CIRCLE('',#104299,0.126999999999998);
#33006=CIRCLE('',#104301,0.127000000000001);
#33007=CIRCLE('',#104303,0.127);
#33008=CIRCLE('',#104304,0.127);
#33009=CIRCLE('',#104305,0.127);
#33010=CIRCLE('',#104307,0.126999999999996);
#33011=CIRCLE('',#104310,0.126999999999998);
#33012=CIRCLE('',#104312,0.127000000000002);
#33013=CIRCLE('',#104314,0.127000000000001);
#33014=CIRCLE('',#104315,0.127);
#33015=CIRCLE('',#104316,0.127);
#33016=CIRCLE('',#104318,0.127);
#33017=CIRCLE('',#104321,0.127000000000001);
#33018=CIRCLE('',#104325,0.126999999999999);
#33019=CIRCLE('',#104326,0.127);
#33020=CIRCLE('',#104328,0.127);
#33021=CIRCLE('',#104330,0.127);
#33022=CIRCLE('',#104331,0.127000000000003);
#33023=CIRCLE('',#104332,0.127000000000001);
#33024=CIRCLE('',#104334,0.126999999999998);
#33025=CIRCLE('',#104337,0.126999999999999);
#33026=CIRCLE('',#104339,0.127);
#33027=CIRCLE('',#104341,0.127000000000003);
#33028=CIRCLE('',#104342,0.126999999999998);
#33029=CIRCLE('',#104343,0.126999999999998);
#33030=CIRCLE('',#104345,0.126999999999998);
#33031=CIRCLE('',#104347,0.127);
#33032=CIRCLE('',#104348,0.127000000000001);
#33033=CIRCLE('',#104349,0.127);
#33034=CIRCLE('',#104351,0.127);
#33035=CIRCLE('',#104354,0.127000000000001);
#33036=CIRCLE('',#104356,0.126999999999997);
#33037=CIRCLE('',#104358,0.126999999999998);
#33038=CIRCLE('',#104359,0.127);
#33039=CIRCLE('',#104360,0.127);
#33040=CIRCLE('',#104362,0.127);
#33041=CIRCLE('',#104365,0.127000000000001);
#33042=CIRCLE('',#104369,0.127000000000001);
#33043=CIRCLE('',#104370,0.127000000000004);
#33044=CIRCLE('',#104372,0.127000000000004);
#33045=CIRCLE('',#104374,0.127000000000004);
#33046=CIRCLE('',#104375,0.126999999999998);
#33047=CIRCLE('',#104376,0.126999999999997);
#33048=CIRCLE('',#104378,0.127);
#33049=CIRCLE('',#104381,0.127000000000001);
#33050=CIRCLE('',#104383,0.127000000000004);
#33051=CIRCLE('',#104385,0.126999999999998);
#33052=CIRCLE('',#104386,0.126999999999997);
#33053=CIRCLE('',#104387,0.127);
#33054=CIRCLE('',#104389,0.126999999999999);
#33055=CIRCLE('',#104391,0.127000000000001);
#33056=CIRCLE('',#104392,0.126999999999996);
#33057=CIRCLE('',#104393,0.127000000000004);
#33058=CIRCLE('',#104395,0.127000000000003);
#33059=CIRCLE('',#104398,0.126999999999999);
#33060=CIRCLE('',#104400,0.127000000000001);
#33061=CIRCLE('',#104402,0.127000000000001);
#33062=CIRCLE('',#104403,0.127000000000004);
#33063=CIRCLE('',#104404,0.127);
#33064=CIRCLE('',#104406,0.127000000000004);
#33065=CIRCLE('',#104409,0.126999999999997);
#33066=CIRCLE('',#104413,0.127000000000001);
#33067=CIRCLE('',#104414,0.127);
#33068=CIRCLE('',#104416,0.127);
#33069=CIRCLE('',#104418,0.126999999999999);
#33070=CIRCLE('',#104419,0.126999999999999);
#33071=CIRCLE('',#104420,0.126999999999998);
#33072=CIRCLE('',#104422,0.127);
#33073=CIRCLE('',#104425,0.127000000000002);
#33074=CIRCLE('',#104427,0.127);
#33075=CIRCLE('',#104429,0.127000000000002);
#33076=CIRCLE('',#104430,0.127000000000002);
#33077=CIRCLE('',#104431,0.127);
#33078=CIRCLE('',#104433,0.126999999999998);
#33079=CIRCLE('',#104435,0.126999999999999);
#33080=CIRCLE('',#104436,0.127);
#33081=CIRCLE('',#104437,0.127000000000003);
#33082=CIRCLE('',#104439,0.126999999999998);
#33083=CIRCLE('',#104442,0.127000000000001);
#33084=CIRCLE('',#104444,0.127000000000001);
#33085=CIRCLE('',#104446,0.127000000000002);
#33086=CIRCLE('',#104447,0.127);
#33087=CIRCLE('',#104448,0.127);
#33088=CIRCLE('',#104450,0.127);
#33089=CIRCLE('',#104453,0.127000000000001);
#33090=CIRCLE('',#104457,0.127);
#33091=CIRCLE('',#104458,0.127000000000001);
#33092=CIRCLE('',#104460,0.127000000000001);
#33093=CIRCLE('',#104462,0.127000000000001);
#33094=CIRCLE('',#104463,0.127000000000001);
#33095=CIRCLE('',#104464,0.127000000000004);
#33096=CIRCLE('',#104466,0.126999999999999);
#33097=CIRCLE('',#104469,0.127000000000001);
#33098=CIRCLE('',#104471,0.126999999999998);
#33099=CIRCLE('',#104473,0.127000000000001);
#33100=CIRCLE('',#104474,0.127000000000001);
#33101=CIRCLE('',#104475,0.127);
#33102=CIRCLE('',#104477,0.126999999999997);
#33103=CIRCLE('',#104479,0.126999999999997);
#33104=CIRCLE('',#104480,0.127000000000003);
#33105=CIRCLE('',#104481,0.127000000000001);
#33106=CIRCLE('',#104483,0.127000000000001);
#33107=CIRCLE('',#104486,0.127);
#33108=CIRCLE('',#104488,0.127);
#33109=CIRCLE('',#104490,0.126999999999998);
#33110=CIRCLE('',#104491,0.127000000000001);
#33111=CIRCLE('',#104492,0.127000000000001);
#33112=CIRCLE('',#104494,0.127000000000001);
#33113=CIRCLE('',#104497,0.127000000000001);
#33114=CIRCLE('',#104501,0.127000000000001);
#33115=CIRCLE('',#104502,0.127);
#33116=CIRCLE('',#104504,0.127);
#33117=CIRCLE('',#104506,0.127);
#33118=CIRCLE('',#104507,0.127000000000002);
#33119=CIRCLE('',#104508,0.126999999999997);
#33120=CIRCLE('',#104510,0.127);
#33121=CIRCLE('',#104513,0.127);
#33122=CIRCLE('',#104515,0.127);
#33123=CIRCLE('',#104517,0.126999999999998);
#33124=CIRCLE('',#104518,0.127000000000001);
#33125=CIRCLE('',#104519,0.126999999999997);
#33126=CIRCLE('',#104521,0.126999999999999);
#33127=CIRCLE('',#104523,0.126999999999998);
#33128=CIRCLE('',#104524,0.126999999999999);
#33129=CIRCLE('',#104525,0.127);
#33130=CIRCLE('',#104527,0.127000000000002);
#33131=CIRCLE('',#104530,0.126999999999999);
#33132=CIRCLE('',#104532,0.127000000000001);
#33133=CIRCLE('',#104534,0.127000000000001);
#33134=CIRCLE('',#104535,0.127);
#33135=CIRCLE('',#104536,0.127);
#33136=CIRCLE('',#104538,0.127);
#33137=CIRCLE('',#104541,0.127000000000003);
#33138=CIRCLE('',#104545,0.127000000000001);
#33139=CIRCLE('',#104546,0.126999999999999);
#33140=CIRCLE('',#104548,0.126999999999999);
#33141=CIRCLE('',#104550,0.126999999999999);
#33142=CIRCLE('',#104551,0.127000000000002);
#33143=CIRCLE('',#104552,0.127000000000003);
#33144=CIRCLE('',#104554,0.127000000000002);
#33145=CIRCLE('',#104557,0.127000000000003);
#33146=CIRCLE('',#104559,0.126999999999999);
#33147=CIRCLE('',#104561,0.126999999999996);
#33148=CIRCLE('',#104562,0.127000000000002);
#33149=CIRCLE('',#104563,0.126999999999999);
#33150=CIRCLE('',#104565,0.127000000000001);
#33151=CIRCLE('',#104567,0.127000000000002);
#33152=CIRCLE('',#104568,0.127);
#33153=CIRCLE('',#104569,0.126999999999999);
#33154=CIRCLE('',#104571,0.127000000000002);
#33155=CIRCLE('',#104574,0.127000000000001);
#33156=CIRCLE('',#104576,0.126999999999997);
#33157=CIRCLE('',#104578,0.127);
#33158=CIRCLE('',#104579,0.126999999999999);
#33159=CIRCLE('',#104580,0.126999999999999);
#33160=CIRCLE('',#104582,0.126999999999999);
#33161=CIRCLE('',#104585,0.127);
#33162=CIRCLE('',#104589,0.126999999999998);
#33163=CIRCLE('',#104590,0.127);
#33164=CIRCLE('',#104592,0.127);
#33165=CIRCLE('',#104594,0.127);
#33166=CIRCLE('',#104595,0.126999999999998);
#33167=CIRCLE('',#104596,0.127);
#33168=CIRCLE('',#104598,0.126999999999999);
#33169=CIRCLE('',#104601,0.127000000000002);
#33170=CIRCLE('',#104603,0.127);
#33171=CIRCLE('',#104605,0.127000000000004);
#33172=CIRCLE('',#104606,0.126999999999998);
#33173=CIRCLE('',#104607,0.127);
#33174=CIRCLE('',#104609,0.127000000000001);
#33175=CIRCLE('',#104611,0.126999999999998);
#33176=CIRCLE('',#104612,0.126999999999997);
#33177=CIRCLE('',#104613,0.127);
#33178=CIRCLE('',#104615,0.127);
#33179=CIRCLE('',#104618,0.127000000000001);
#33180=CIRCLE('',#104620,0.126999999999999);
#33181=CIRCLE('',#104622,0.126999999999998);
#33182=CIRCLE('',#104623,0.127);
#33183=CIRCLE('',#104624,0.127);
#33184=CIRCLE('',#104626,0.127);
#33185=CIRCLE('',#104629,0.127);
#33186=CIRCLE('',#104632,59.0285554514622);
#33187=CIRCLE('',#104633,0.127000000000002);
#33188=CIRCLE('',#104634,58.9208533432504);
#33189=CIRCLE('',#104635,0.127000000000002);
#33190=CIRCLE('',#104637,62.9541466567496);
#33191=CIRCLE('',#104638,0.127000000000002);
#33192=CIRCLE('',#104639,62.8464445485378);
#33193=CIRCLE('',#104640,0.127000000000002);
#33194=CIRCLE('',#104642,59.0285554514622);
#33195=CIRCLE('',#104643,0.127000000000002);
#33196=CIRCLE('',#104644,58.9208533432504);
#33197=CIRCLE('',#104645,0.127000000000002);
#33198=CIRCLE('',#104647,62.9541466567496);
#33199=CIRCLE('',#104648,0.127000000000002);
#33200=CIRCLE('',#104649,62.8464445485378);
#33201=CIRCLE('',#104650,0.127000000000002);
#33202=CIRCLE('',#104651,62.9541466567496);
#33203=CIRCLE('',#104653,58.2189663438286);
#33204=CIRCLE('',#104654,0.635);
#33205=CIRCLE('',#104655,57.6804558027693);
#33206=CIRCLE('',#104656,57.6804558027693);
#33207=CIRCLE('',#104658,58.8470884664677);
#33208=CIRCLE('',#104659,0.635);
#33209=CIRCLE('',#104660,58.3085779254084);
#33210=CIRCLE('',#104662,63.5664220745916);
#33211=CIRCLE('',#104663,0.635);
#33212=CIRCLE('',#104664,63.0279115335323);
#33213=CIRCLE('',#104665,63.0279115335323);
#33214=CIRCLE('',#104667,64.1945441972308);
#33215=CIRCLE('',#104668,0.635);
#33216=CIRCLE('',#104669,63.6560336561714);
#33217=CIRCLE('',#104671,65.);
#33218=CIRCLE('',#104672,65.);
#33219=CIRCLE('',#104675,62.9541466567496);
#33220=CIRCLE('',#104676,62.4089800241499);
#33221=CIRCLE('',#104677,62.9541466567496);
#33222=CIRCLE('',#104678,62.4089800241499);
#33223=CIRCLE('',#104679,62.9541466567496);
#33224=CIRCLE('',#104680,62.4089800241499);
#33225=CIRCLE('',#104681,62.9541466567497);
#33226=CIRCLE('',#104682,62.4089800241499);
#33227=CIRCLE('',#104683,62.9541466567496);
#33228=CIRCLE('',#104684,62.4089800241499);
#33229=CIRCLE('',#104685,62.9541466567496);
#33230=CIRCLE('',#104686,62.4089800241499);
#33231=CIRCLE('',#104687,62.9541466567497);
#33232=CIRCLE('',#104688,62.4089800241499);
#33233=CIRCLE('',#104689,62.9541466567497);
#33234=CIRCLE('',#104690,62.4089800241499);
#33235=CIRCLE('',#104691,62.9541466567496);
#33236=CIRCLE('',#104692,62.4089800241499);
#33237=CIRCLE('',#104693,62.9541466567497);
#33238=CIRCLE('',#104694,62.4089800241499);
#33239=CIRCLE('',#104695,62.9541466567496);
#33240=CIRCLE('',#104696,62.4089800241499);
#33241=CIRCLE('',#104697,62.9541466567497);
#33242=CIRCLE('',#104698,62.4089800241499);
#33243=CIRCLE('',#104699,62.9541466567497);
#33244=CIRCLE('',#104700,62.4089800241499);
#33245=CIRCLE('',#104701,62.9541466567496);
#33246=CIRCLE('',#104702,62.4089800241499);
#33247=CIRCLE('',#104703,62.9541466567497);
#33248=CIRCLE('',#104704,62.4089800241499);
#33249=CIRCLE('',#104705,62.9541466567496);
#33250=CIRCLE('',#104706,62.4089800241499);
#33251=CIRCLE('',#104707,62.9541466567497);
#33252=CIRCLE('',#104708,62.4089800241499);
#33253=CIRCLE('',#104709,62.9541466567497);
#33254=CIRCLE('',#104710,62.4089800241499);
#33255=CIRCLE('',#104711,62.9541466567496);
#33256=CIRCLE('',#104712,62.4089800241499);
#33257=CIRCLE('',#104713,62.9541466567496);
#33258=CIRCLE('',#104714,62.4089800241499);
#33259=CIRCLE('',#104715,62.9541466567496);
#33260=CIRCLE('',#104716,62.4089800241499);
#33261=CIRCLE('',#104717,62.9541466567496);
#33262=CIRCLE('',#104718,62.4089800241499);
#33263=CIRCLE('',#104719,62.9541466567497);
#33264=CIRCLE('',#104720,62.4089800241499);
#33265=CIRCLE('',#104721,62.9541466567497);
#33266=CIRCLE('',#104722,62.4089800241499);
#33267=CIRCLE('',#104723,62.9541466567496);
#33268=CIRCLE('',#104724,62.4089800241499);
#33269=CIRCLE('',#104725,62.9541466567496);
#33270=CIRCLE('',#104726,62.4089800241499);
#33271=CIRCLE('',#104727,62.9541466567496);
#33272=CIRCLE('',#104728,62.4089800241499);
#33273=CIRCLE('',#104729,62.9541466567497);
#33274=CIRCLE('',#104730,62.4089800241499);
#33275=CIRCLE('',#104731,62.9541466567496);
#33276=CIRCLE('',#104732,62.4089800241499);
#33277=CIRCLE('',#104733,62.9541466567497);
#33278=CIRCLE('',#104734,62.4089800241499);
#33279=CIRCLE('',#104735,62.4089800241499);
#33280=CIRCLE('',#104736,62.9541466567497);
#33281=CIRCLE('',#104737,62.4089800241499);
#33282=CIRCLE('',#104738,62.9541466567496);
#33283=CIRCLE('',#104739,62.4089800241499);
#33284=CIRCLE('',#104740,62.9541466567496);
#33285=CIRCLE('',#104741,62.4089800241499);
#33286=CIRCLE('',#104742,62.9541466567496);
#33287=CIRCLE('',#104743,62.4089800241499);
#33288=CIRCLE('',#104744,62.9541466567497);
#33289=CIRCLE('',#104745,62.4089800241499);
#33290=CIRCLE('',#104746,62.9541466567496);
#33291=CIRCLE('',#104747,62.4089800241499);
#33292=CIRCLE('',#104748,62.9541466567497);
#33293=CIRCLE('',#104749,62.4089800241499);
#33294=CIRCLE('',#104750,62.9541466567497);
#33295=CIRCLE('',#104751,62.4089800241499);
#33296=CIRCLE('',#104752,62.9541466567497);
#33297=CIRCLE('',#104753,62.4089800241499);
#33298=CIRCLE('',#104754,62.9541466567496);
#33299=CIRCLE('',#104755,62.4089800241499);
#33300=CIRCLE('',#104756,62.9541466567496);
#33301=CIRCLE('',#104757,62.4089800241499);
#33302=CIRCLE('',#104758,62.9541466567496);
#33303=CIRCLE('',#104759,62.4089800241499);
#33304=CIRCLE('',#104760,62.9541466567497);
#33305=CIRCLE('',#104761,62.4089800241499);
#33306=CIRCLE('',#104762,62.9541466567496);
#33307=CIRCLE('',#104763,62.4089800241499);
#33308=CIRCLE('',#104764,62.4089800241499);
#33309=CIRCLE('',#104765,62.9541466567497);
#33310=CIRCLE('',#104766,62.4089800241499);
#33311=CIRCLE('',#104767,62.9541466567497);
#33312=CIRCLE('',#104768,62.4089800241499);
#33313=CIRCLE('',#104769,62.9541466567497);
#33314=CIRCLE('',#104770,62.4089800241499);
#33315=CIRCLE('',#104771,62.9541466567497);
#33316=CIRCLE('',#104772,62.4089800241499);
#33317=CIRCLE('',#104773,62.9541466567497);
#33318=CIRCLE('',#104774,62.4089800241499);
#33319=CIRCLE('',#104775,62.9541466567496);
#33320=CIRCLE('',#104776,62.4089800241499);
#33321=CIRCLE('',#104777,62.9541466567496);
#33322=CIRCLE('',#104778,62.4089800241499);
#33323=CIRCLE('',#104779,62.9541466567496);
#33324=CIRCLE('',#104780,62.4089800241499);
#33325=CIRCLE('',#104781,62.9541466567497);
#33326=CIRCLE('',#104782,62.4089800241499);
#33327=CIRCLE('',#104783,62.9541466567496);
#33328=CIRCLE('',#104784,62.4089800241499);
#33329=CIRCLE('',#104785,62.9541466567497);
#33330=CIRCLE('',#104786,62.4089800241499);
#33331=CIRCLE('',#104787,62.9541466567497);
#33332=CIRCLE('',#104788,62.4089800241499);
#33333=CIRCLE('',#104789,62.9541466567497);
#33334=CIRCLE('',#104790,62.4089800241499);
#33335=CIRCLE('',#104791,62.9541466567497);
#33336=CIRCLE('',#104792,62.4089800241499);
#33337=CIRCLE('',#104794,59.4660199758502);
#33338=CIRCLE('',#104795,58.9208533432504);
#33339=CIRCLE('',#104796,59.4660199758502);
#33340=CIRCLE('',#104797,58.9208533432504);
#33341=CIRCLE('',#104798,59.4660199758502);
#33342=CIRCLE('',#104799,58.9208533432504);
#33343=CIRCLE('',#104800,59.4660199758502);
#33344=CIRCLE('',#104801,58.9208533432504);
#33345=CIRCLE('',#104802,59.4660199758502);
#33346=CIRCLE('',#104803,58.9208533432504);
#33347=CIRCLE('',#104804,59.4660199758502);
#33348=CIRCLE('',#104805,58.9208533432504);
#33349=CIRCLE('',#104806,59.4660199758502);
#33350=CIRCLE('',#104807,58.9208533432504);
#33351=CIRCLE('',#104808,59.4660199758502);
#33352=CIRCLE('',#104809,58.9208533432504);
#33353=CIRCLE('',#104810,59.4660199758502);
#33354=CIRCLE('',#104811,58.9208533432504);
#33355=CIRCLE('',#104812,59.4660199758502);
#33356=CIRCLE('',#104813,58.9208533432504);
#33357=CIRCLE('',#104814,59.4660199758502);
#33358=CIRCLE('',#104815,58.9208533432504);
#33359=CIRCLE('',#104816,59.4660199758502);
#33360=CIRCLE('',#104817,58.9208533432504);
#33361=CIRCLE('',#104818,59.4660199758502);
#33362=CIRCLE('',#104819,58.9208533432504);
#33363=CIRCLE('',#104820,59.4660199758502);
#33364=CIRCLE('',#104821,58.9208533432504);
#33365=CIRCLE('',#104822,59.4660199758502);
#33366=CIRCLE('',#104823,58.9208533432504);
#33367=CIRCLE('',#104824,59.4660199758502);
#33368=CIRCLE('',#104825,58.9208533432504);
#33369=CIRCLE('',#104826,59.4660199758502);
#33370=CIRCLE('',#104827,58.9208533432504);
#33371=CIRCLE('',#104828,59.4660199758502);
#33372=CIRCLE('',#104829,58.9208533432504);
#33373=CIRCLE('',#104830,59.4660199758502);
#33374=CIRCLE('',#104831,58.9208533432504);
#33375=CIRCLE('',#104832,59.4660199758502);
#33376=CIRCLE('',#104833,58.9208533432504);
#33377=CIRCLE('',#104834,59.4660199758502);
#33378=CIRCLE('',#104835,58.9208533432504);
#33379=CIRCLE('',#104836,59.4660199758502);
#33380=CIRCLE('',#104837,58.9208533432504);
#33381=CIRCLE('',#104838,59.4660199758502);
#33382=CIRCLE('',#104839,58.9208533432504);
#33383=CIRCLE('',#104840,59.4660199758502);
#33384=CIRCLE('',#104841,58.9208533432504);
#33385=CIRCLE('',#104842,59.4660199758502);
#33386=CIRCLE('',#104843,58.9208533432504);
#33387=CIRCLE('',#104844,59.4660199758502);
#33388=CIRCLE('',#104845,58.9208533432504);
#33389=CIRCLE('',#104846,59.4660199758502);
#33390=CIRCLE('',#104847,58.9208533432504);
#33391=CIRCLE('',#104848,59.4660199758502);
#33392=CIRCLE('',#104849,58.9208533432504);
#33393=CIRCLE('',#104850,59.4660199758502);
#33394=CIRCLE('',#104851,58.9208533432504);
#33395=CIRCLE('',#104852,59.4660199758502);
#33396=CIRCLE('',#104853,58.9208533432504);
#33397=CIRCLE('',#104854,58.9208533432504);
#33398=CIRCLE('',#104855,59.4660199758502);
#33399=CIRCLE('',#104856,58.9208533432504);
#33400=CIRCLE('',#104857,59.4660199758502);
#33401=CIRCLE('',#104858,58.9208533432504);
#33402=CIRCLE('',#104859,59.4660199758502);
#33403=CIRCLE('',#104860,58.9208533432504);
#33404=CIRCLE('',#104861,59.4660199758502);
#33405=CIRCLE('',#104862,58.9208533432504);
#33406=CIRCLE('',#104863,59.4660199758502);
#33407=CIRCLE('',#104864,58.9208533432504);
#33408=CIRCLE('',#104865,59.4660199758502);
#33409=CIRCLE('',#104866,58.9208533432504);
#33410=CIRCLE('',#104867,59.4660199758502);
#33411=CIRCLE('',#104868,58.9208533432504);
#33412=CIRCLE('',#104869,59.4660199758502);
#33413=CIRCLE('',#104870,58.9208533432504);
#33414=CIRCLE('',#104871,59.4660199758502);
#33415=CIRCLE('',#104872,58.9208533432504);
#33416=CIRCLE('',#104873,59.4660199758502);
#33417=CIRCLE('',#104874,58.9208533432504);
#33418=CIRCLE('',#104875,59.4660199758502);
#33419=CIRCLE('',#104876,58.9208533432504);
#33420=CIRCLE('',#104877,59.4660199758502);
#33421=CIRCLE('',#104878,58.9208533432504);
#33422=CIRCLE('',#104879,59.4660199758502);
#33423=CIRCLE('',#104880,58.9208533432504);
#33424=CIRCLE('',#104881,59.4660199758502);
#33425=CIRCLE('',#104882,58.9208533432504);
#33426=CIRCLE('',#104883,59.4660199758502);
#33427=CIRCLE('',#104884,59.4660199758502);
#33428=CIRCLE('',#104885,58.9208533432504);
#33429=CIRCLE('',#104886,59.4660199758502);
#33430=CIRCLE('',#104887,58.9208533432504);
#33431=CIRCLE('',#104888,59.4660199758502);
#33432=CIRCLE('',#104889,58.9208533432504);
#33433=CIRCLE('',#104890,59.4660199758502);
#33434=CIRCLE('',#104891,58.9208533432504);
#33435=CIRCLE('',#104892,59.4660199758502);
#33436=CIRCLE('',#104893,58.9208533432504);
#33437=CIRCLE('',#104894,59.4660199758502);
#33438=CIRCLE('',#104895,58.9208533432504);
#33439=CIRCLE('',#104896,59.4660199758502);
#33440=CIRCLE('',#104897,58.9208533432504);
#33441=CIRCLE('',#104898,59.4660199758502);
#33442=CIRCLE('',#104899,58.9208533432504);
#33443=CIRCLE('',#104900,59.4660199758502);
#33444=CIRCLE('',#104901,58.9208533432504);
#33445=CIRCLE('',#104902,59.4660199758502);
#33446=CIRCLE('',#104903,58.9208533432504);
#33447=CIRCLE('',#104904,59.4660199758502);
#33448=CIRCLE('',#104905,58.9208533432504);
#33449=CIRCLE('',#104906,59.4660199758502);
#33450=CIRCLE('',#104907,58.9208533432504);
#33451=CIRCLE('',#104908,59.4660199758502);
#33452=CIRCLE('',#104909,58.9208533432504);
#33453=CIRCLE('',#104910,59.4660199758502);
#33454=CIRCLE('',#104911,58.9208533432504);
#33455=CIRCLE('',#104912,59.4660199758502);
#33456=CIRCLE('',#104914,56.875);
#33457=CIRCLE('',#104915,56.875);
#33458=CIRCLE('',#104917,56.875);
#33459=CIRCLE('',#104919,60.4792282238308);
#33460=CIRCLE('',#104920,60.0045305169095);
#33461=CIRCLE('',#104921,60.4792282238308);
#33462=CIRCLE('',#104922,60.4792282238308);
#33463=CIRCLE('',#104924,60.6419265158129);
#33464=CIRCLE('',#104926,61.0131030316259);
#33465=CIRCLE('',#104927,60.8618969683742);
#33466=CIRCLE('',#104929,61.3957717761693);
#33467=CIRCLE('',#104930,61.2330734841871);
#33468=CIRCLE('',#104931,61.3957717761693);
#33469=CIRCLE('',#104932,61.3957717761693);
#33470=CIRCLE('',#104934,61.8704694830905);
#33471=CIRCLE('',#104936,0.635007073208622);
#33472=CIRCLE('',#104937,0.635007073208628);
#33473=CIRCLE('',#104948,60.0045305169095);
#33474=CIRCLE('',#104949,60.4792282238308);
#33475=CIRCLE('',#104950,60.4792282238308);
#33476=CIRCLE('',#104951,60.4792282238308);
#33477=CIRCLE('',#104953,60.6419265158129);
#33478=CIRCLE('',#104955,60.8618969683742);
#33479=CIRCLE('',#104956,61.0131030316259);
#33480=CIRCLE('',#104958,61.2330734841871);
#33481=CIRCLE('',#104959,61.3957717761693);
#33482=CIRCLE('',#104960,61.3957717761693);
#33483=CIRCLE('',#104961,61.3957717761693);
#33484=CIRCLE('',#104963,61.8704694830905);
#33485=CIRCLE('',#104965,0.635007073208604);
#33486=CIRCLE('',#104966,0.635007073208616);
#33487=CIRCLE('',#104977,60.0045305169095);
#33488=CIRCLE('',#104978,60.4792282238308);
#33489=CIRCLE('',#104979,60.4792282238308);
#33490=CIRCLE('',#104980,60.4792282238308);
#33491=CIRCLE('',#104982,60.6419265158129);
#33492=CIRCLE('',#104984,60.8618969683742);
#33493=CIRCLE('',#104985,61.0131030316259);
#33494=CIRCLE('',#104987,61.2330734841871);
#33495=CIRCLE('',#104988,61.3957717761693);
#33496=CIRCLE('',#104989,61.3957717761693);
#33497=CIRCLE('',#104990,61.3957717761693);
#33498=CIRCLE('',#104992,61.8704694830905);
#33499=CIRCLE('',#104994,0.635007073208621);
#33500=CIRCLE('',#104995,0.635007073208653);
#33501=CIRCLE('',#105006,60.0045305169095);
#33502=CIRCLE('',#105007,60.4792282238308);
#33503=CIRCLE('',#105008,60.4792282238308);
#33504=CIRCLE('',#105009,60.4792282238308);
#33505=CIRCLE('',#105011,60.6419265158129);
#33506=CIRCLE('',#105013,60.8618969683742);
#33507=CIRCLE('',#105014,61.0131030316259);
#33508=CIRCLE('',#105016,61.2330734841871);
#33509=CIRCLE('',#105017,61.3957717761693);
#33510=CIRCLE('',#105018,61.3957717761693);
#33511=CIRCLE('',#105019,61.3957717761693);
#33512=CIRCLE('',#105021,61.8704694830905);
#33513=CIRCLE('',#105023,0.635007073208651);
#33514=CIRCLE('',#105024,0.63500707320859);
#33515=CIRCLE('',#105035,60.0045305169095);
#33516=CIRCLE('',#105036,60.4792282238308);
#33517=CIRCLE('',#105037,60.4792282238308);
#33518=CIRCLE('',#105038,60.4792282238308);
#33519=CIRCLE('',#105040,60.6419265158129);
#33520=CIRCLE('',#105042,60.8618969683742);
#33521=CIRCLE('',#105043,61.0131030316259);
#33522=CIRCLE('',#105045,61.2330734841871);
#33523=CIRCLE('',#105046,61.3957717761693);
#33524=CIRCLE('',#105047,61.3957717761693);
#33525=CIRCLE('',#105048,61.3957717761693);
#33526=CIRCLE('',#105050,61.8704694830905);
#33527=CIRCLE('',#105052,0.63500707320864);
#33528=CIRCLE('',#105053,0.635007073208627);
#33529=CIRCLE('',#105064,60.0045305169095);
#33530=CIRCLE('',#105065,60.4792282238308);
#33531=CIRCLE('',#105066,60.4792282238308);
#33532=CIRCLE('',#105067,60.4792282238308);
#33533=CIRCLE('',#105069,60.6419265158129);
#33534=CIRCLE('',#105071,60.8618969683742);
#33535=CIRCLE('',#105072,61.0131030316259);
#33536=CIRCLE('',#105074,61.2330734841871);
#33537=CIRCLE('',#105075,61.3957717761693);
#33538=CIRCLE('',#105076,61.3957717761693);
#33539=CIRCLE('',#105077,61.3957717761693);
#33540=CIRCLE('',#105079,61.8704694830905);
#33541=CIRCLE('',#105081,0.635007073208625);
#33542=CIRCLE('',#105082,0.635007073208636);
#33543=CIRCLE('',#105093,60.0045305169095);
#33544=CIRCLE('',#105094,60.4792282238308);
#33545=CIRCLE('',#105095,60.4792282238308);
#33546=CIRCLE('',#105096,60.4792282238308);
#33547=CIRCLE('',#105098,60.6419265158129);
#33548=CIRCLE('',#105100,60.8618969683742);
#33549=CIRCLE('',#105101,61.0131030316259);
#33550=CIRCLE('',#105103,61.2330734841871);
#33551=CIRCLE('',#105104,61.3957717761693);
#33552=CIRCLE('',#105105,61.3957717761693);
#33553=CIRCLE('',#105106,61.3957717761693);
#33554=CIRCLE('',#105108,61.8704694830905);
#33555=CIRCLE('',#105110,0.635007073208613);
#33556=CIRCLE('',#105111,0.635007073208626);
#33557=CIRCLE('',#105122,60.0045305169095);
#33558=CIRCLE('',#105123,60.4792282238308);
#33559=CIRCLE('',#105124,60.4792282238308);
#33560=CIRCLE('',#105125,60.4792282238308);
#33561=CIRCLE('',#105127,60.6419265158129);
#33562=CIRCLE('',#105129,60.8618969683742);
#33563=CIRCLE('',#105130,61.0131030316259);
#33564=CIRCLE('',#105132,61.2330734841871);
#33565=CIRCLE('',#105133,61.3957717761693);
#33566=CIRCLE('',#105134,61.3957717761693);
#33567=CIRCLE('',#105135,61.3957717761693);
#33568=CIRCLE('',#105137,61.8704694830905);
#33569=CIRCLE('',#105139,0.635007073208636);
#33570=CIRCLE('',#105140,0.635007073208635);
#33571=CIRCLE('',#105151,60.0045305169095);
#33572=CIRCLE('',#105152,60.4792282238308);
#33573=CIRCLE('',#105153,60.4792282238308);
#33574=CIRCLE('',#105154,60.4792282238308);
#33575=CIRCLE('',#105156,60.6419265158129);
#33576=CIRCLE('',#105158,60.8618969683742);
#33577=CIRCLE('',#105159,61.0131030316259);
#33578=CIRCLE('',#105161,61.2330734841871);
#33579=CIRCLE('',#105162,61.3957717761693);
#33580=CIRCLE('',#105163,61.3957717761693);
#33581=CIRCLE('',#105164,61.3957717761693);
#33582=CIRCLE('',#105166,61.8704694830905);
#33583=CIRCLE('',#105168,0.635007073208616);
#33584=CIRCLE('',#105169,0.635007073208608);
#33585=CIRCLE('',#105180,60.0045305169095);
#33586=CIRCLE('',#105181,60.4792282238308);
#33587=CIRCLE('',#105182,60.4792282238308);
#33588=CIRCLE('',#105183,60.4792282238308);
#33589=CIRCLE('',#105185,60.6419265158129);
#33590=CIRCLE('',#105187,60.8618969683742);
#33591=CIRCLE('',#105188,61.0131030316259);
#33592=CIRCLE('',#105190,61.2330734841871);
#33593=CIRCLE('',#105191,61.3957717761693);
#33594=CIRCLE('',#105192,61.3957717761693);
#33595=CIRCLE('',#105193,61.3957717761693);
#33596=CIRCLE('',#105195,61.8704694830905);
#33597=CIRCLE('',#105197,0.635007073208567);
#33598=CIRCLE('',#105198,0.635007073208631);
#33599=CIRCLE('',#105209,60.0045305169095);
#33600=CIRCLE('',#105210,60.4792282238308);
#33601=CIRCLE('',#105211,60.4792282238308);
#33602=CIRCLE('',#105212,60.4792282238308);
#33603=CIRCLE('',#105214,60.6419265158129);
#33604=CIRCLE('',#105216,60.8618969683742);
#33605=CIRCLE('',#105217,61.0131030316259);
#33606=CIRCLE('',#105219,61.2330734841871);
#33607=CIRCLE('',#105220,61.3957717761693);
#33608=CIRCLE('',#105221,61.3957717761693);
#33609=CIRCLE('',#105222,61.3957717761693);
#33610=CIRCLE('',#105224,61.8704694830905);
#33611=CIRCLE('',#105226,0.635007073208609);
#33612=CIRCLE('',#105227,0.635007073208634);
#33613=CIRCLE('',#105238,60.0045305169095);
#33614=CIRCLE('',#105239,60.4792282238308);
#33615=CIRCLE('',#105240,60.4792282238308);
#33616=CIRCLE('',#105241,60.4792282238308);
#33617=CIRCLE('',#105243,60.6419265158129);
#33618=CIRCLE('',#105245,60.8618969683742);
#33619=CIRCLE('',#105246,61.0131030316259);
#33620=CIRCLE('',#105248,61.2330734841871);
#33621=CIRCLE('',#105249,61.3957717761693);
#33622=CIRCLE('',#105250,61.3957717761693);
#33623=CIRCLE('',#105251,61.3957717761693);
#33624=CIRCLE('',#105253,61.8704694830905);
#33625=CIRCLE('',#105255,0.63500707320864);
#33626=CIRCLE('',#105256,0.635007073208652);
#33627=CIRCLE('',#105267,60.0045305169095);
#33628=CIRCLE('',#105268,60.4792282238308);
#33629=CIRCLE('',#105269,60.4792282238308);
#33630=CIRCLE('',#105270,60.4792282238308);
#33631=CIRCLE('',#105272,60.6419265158129);
#33632=CIRCLE('',#105274,60.8618969683742);
#33633=CIRCLE('',#105275,61.0131030316259);
#33634=CIRCLE('',#105277,61.2330734841871);
#33635=CIRCLE('',#105278,61.3957717761693);
#33636=CIRCLE('',#105279,61.3957717761693);
#33637=CIRCLE('',#105280,61.3957717761693);
#33638=CIRCLE('',#105282,61.8704694830905);
#33639=CIRCLE('',#105284,0.635007073208623);
#33640=CIRCLE('',#105285,0.635007073208637);
#33641=CIRCLE('',#105296,60.0045305169095);
#33642=CIRCLE('',#105297,60.4792282238308);
#33643=CIRCLE('',#105298,60.4792282238308);
#33644=CIRCLE('',#105299,60.4792282238308);
#33645=CIRCLE('',#105301,60.6419265158129);
#33646=CIRCLE('',#105303,60.8618969683742);
#33647=CIRCLE('',#105304,61.0131030316259);
#33648=CIRCLE('',#105306,61.2330734841871);
#33649=CIRCLE('',#105307,61.3957717761693);
#33650=CIRCLE('',#105308,61.3957717761693);
#33651=CIRCLE('',#105309,61.3957717761693);
#33652=CIRCLE('',#105311,61.8704694830905);
#33653=CIRCLE('',#105313,0.635007073208589);
#33654=CIRCLE('',#105314,0.635007073208633);
#33655=CIRCLE('',#105325,60.0045305169095);
#33656=CIRCLE('',#105326,60.4792282238308);
#33657=CIRCLE('',#105327,60.4792282238308);
#33658=CIRCLE('',#105328,60.4792282238308);
#33659=CIRCLE('',#105330,60.6419265158129);
#33660=CIRCLE('',#105332,60.8618969683742);
#33661=CIRCLE('',#105333,61.0131030316259);
#33662=CIRCLE('',#105335,61.2330734841871);
#33663=CIRCLE('',#105336,61.3957717761693);
#33664=CIRCLE('',#105337,61.3957717761693);
#33665=CIRCLE('',#105338,61.3957717761693);
#33666=CIRCLE('',#105340,61.8704694830905);
#33667=CIRCLE('',#105342,0.635007073208619);
#33668=CIRCLE('',#105343,0.635007073208628);
#33669=CIRCLE('',#105354,60.0045305169095);
#33670=CIRCLE('',#105355,60.4792282238308);
#33671=CIRCLE('',#105356,60.4792282238308);
#33672=CIRCLE('',#105357,60.4792282238308);
#33673=CIRCLE('',#105359,60.6419265158129);
#33674=CIRCLE('',#105361,60.8618969683742);
#33675=CIRCLE('',#105362,61.0131030316259);
#33676=CIRCLE('',#105364,61.2330734841871);
#33677=CIRCLE('',#105365,61.3957717761693);
#33678=CIRCLE('',#105366,61.3957717761693);
#33679=CIRCLE('',#105367,61.3957717761693);
#33680=CIRCLE('',#105369,61.8704694830905);
#33681=CIRCLE('',#105371,0.635007073208656);
#33682=CIRCLE('',#105372,0.635007073208614);
#33683=CIRCLE('',#105383,60.0045305169095);
#33684=CIRCLE('',#105384,60.4792282238308);
#33685=CIRCLE('',#105385,60.4792282238308);
#33686=CIRCLE('',#105386,60.4792282238308);
#33687=CIRCLE('',#105388,60.6419265158129);
#33688=CIRCLE('',#105390,60.8618969683742);
#33689=CIRCLE('',#105391,61.0131030316259);
#33690=CIRCLE('',#105393,61.2330734841871);
#33691=CIRCLE('',#105394,61.3957717761693);
#33692=CIRCLE('',#105395,61.3957717761693);
#33693=CIRCLE('',#105396,61.3957717761693);
#33694=CIRCLE('',#105398,61.8704694830905);
#33695=CIRCLE('',#105400,0.635007073208594);
#33696=CIRCLE('',#105401,0.635007073208644);
#33697=CIRCLE('',#105412,60.0045305169095);
#33698=CIRCLE('',#105413,60.4792282238308);
#33699=CIRCLE('',#105414,60.4792282238308);
#33700=CIRCLE('',#105415,60.4792282238308);
#33701=CIRCLE('',#105417,60.6419265158129);
#33702=CIRCLE('',#105419,60.8618969683742);
#33703=CIRCLE('',#105420,61.0131030316259);
#33704=CIRCLE('',#105422,61.2330734841871);
#33705=CIRCLE('',#105423,61.3957717761693);
#33706=CIRCLE('',#105424,61.3957717761693);
#33707=CIRCLE('',#105425,61.3957717761693);
#33708=CIRCLE('',#105427,61.8704694830905);
#33709=CIRCLE('',#105429,0.635007073208621);
#33710=CIRCLE('',#105430,0.635007073208619);
#33711=CIRCLE('',#105441,60.0045305169095);
#33712=CIRCLE('',#105442,60.4792282238308);
#33713=CIRCLE('',#105443,60.4792282238308);
#33714=CIRCLE('',#105444,60.4792282238308);
#33715=CIRCLE('',#105446,60.6419265158129);
#33716=CIRCLE('',#105448,60.8618969683742);
#33717=CIRCLE('',#105449,61.0131030316259);
#33718=CIRCLE('',#105451,61.2330734841871);
#33719=CIRCLE('',#105452,61.3957717761693);
#33720=CIRCLE('',#105453,61.3957717761693);
#33721=CIRCLE('',#105454,61.3957717761693);
#33722=CIRCLE('',#105456,61.8704694830905);
#33723=CIRCLE('',#105458,0.635007073208605);
#33724=CIRCLE('',#105459,0.635007073208611);
#33725=CIRCLE('',#105470,60.0045305169095);
#33726=CIRCLE('',#105471,60.4792282238308);
#33727=CIRCLE('',#105472,60.4792282238308);
#33728=CIRCLE('',#105473,60.4792282238308);
#33729=CIRCLE('',#105475,60.6419265158129);
#33730=CIRCLE('',#105477,60.8618969683742);
#33731=CIRCLE('',#105478,61.0131030316259);
#33732=CIRCLE('',#105480,61.2330734841871);
#33733=CIRCLE('',#105481,61.3957717761693);
#33734=CIRCLE('',#105482,61.3957717761693);
#33735=CIRCLE('',#105483,61.3957717761693);
#33736=CIRCLE('',#105485,61.8704694830905);
#33737=CIRCLE('',#105487,0.635007073208634);
#33738=CIRCLE('',#105488,0.63500707320863);
#33739=CIRCLE('',#105499,60.0045305169095);
#33740=CIRCLE('',#105500,60.4792282238308);
#33741=CIRCLE('',#105501,60.4792282238308);
#33742=CIRCLE('',#105502,60.4792282238308);
#33743=CIRCLE('',#105504,60.6419265158129);
#33744=CIRCLE('',#105506,60.8618969683742);
#33745=CIRCLE('',#105507,61.0131030316259);
#33746=CIRCLE('',#105509,61.2330734841871);
#33747=CIRCLE('',#105510,61.3957717761693);
#33748=CIRCLE('',#105511,61.3957717761693);
#33749=CIRCLE('',#105512,61.3957717761693);
#33750=CIRCLE('',#105514,61.8704694830905);
#33751=CIRCLE('',#105516,0.635007073208654);
#33752=CIRCLE('',#105517,0.635007073208608);
#33753=CIRCLE('',#105528,60.0045305169095);
#33754=CIRCLE('',#105529,60.4792282238308);
#33755=CIRCLE('',#105530,60.4792282238308);
#33756=CIRCLE('',#105531,60.4792282238308);
#33757=CIRCLE('',#105533,60.6419265158129);
#33758=CIRCLE('',#105535,60.8618969683742);
#33759=CIRCLE('',#105536,61.0131030316259);
#33760=CIRCLE('',#105538,61.2330734841871);
#33761=CIRCLE('',#105539,61.3957717761693);
#33762=CIRCLE('',#105540,61.3957717761693);
#33763=CIRCLE('',#105541,61.3957717761693);
#33764=CIRCLE('',#105543,61.8704694830905);
#33765=CIRCLE('',#105545,0.6350070732086);
#33766=CIRCLE('',#105546,0.635007073208599);
#33767=CIRCLE('',#105557,60.0045305169095);
#33768=CIRCLE('',#105558,60.4792282238308);
#33769=CIRCLE('',#105559,60.4792282238308);
#33770=CIRCLE('',#105560,60.4792282238308);
#33771=CIRCLE('',#105562,60.6419265158129);
#33772=CIRCLE('',#105564,60.8618969683742);
#33773=CIRCLE('',#105565,61.0131030316259);
#33774=CIRCLE('',#105567,61.2330734841871);
#33775=CIRCLE('',#105568,61.3957717761693);
#33776=CIRCLE('',#105569,61.3957717761693);
#33777=CIRCLE('',#105570,61.3957717761693);
#33778=CIRCLE('',#105572,61.8704694830905);
#33779=CIRCLE('',#105574,0.635007073208643);
#33780=CIRCLE('',#105575,0.635007073208631);
#33781=CIRCLE('',#105586,60.0045305169095);
#33782=CIRCLE('',#105587,60.4792282238308);
#33783=CIRCLE('',#105588,60.4792282238308);
#33784=CIRCLE('',#105589,60.4792282238308);
#33785=CIRCLE('',#105591,60.6419265158129);
#33786=CIRCLE('',#105593,60.8618969683742);
#33787=CIRCLE('',#105594,61.0131030316259);
#33788=CIRCLE('',#105596,61.2330734841871);
#33789=CIRCLE('',#105597,61.3957717761693);
#33790=CIRCLE('',#105598,61.3957717761693);
#33791=CIRCLE('',#105599,61.3957717761693);
#33792=CIRCLE('',#105601,61.8704694830905);
#33793=CIRCLE('',#105603,0.635007073208614);
#33794=CIRCLE('',#105604,0.635007073208602);
#33795=CIRCLE('',#105615,60.0045305169095);
#33796=CIRCLE('',#105616,60.4792282238308);
#33797=CIRCLE('',#105617,60.4792282238308);
#33798=CIRCLE('',#105618,60.4792282238308);
#33799=CIRCLE('',#105620,60.6419265158129);
#33800=CIRCLE('',#105622,60.8618969683742);
#33801=CIRCLE('',#105623,61.0131030316259);
#33802=CIRCLE('',#105625,61.2330734841871);
#33803=CIRCLE('',#105626,61.3957717761693);
#33804=CIRCLE('',#105627,61.3957717761693);
#33805=CIRCLE('',#105628,61.3957717761693);
#33806=CIRCLE('',#105630,61.8704694830905);
#33807=CIRCLE('',#105632,0.635007073208624);
#33808=CIRCLE('',#105633,0.635007073208626);
#33809=CIRCLE('',#105644,60.0045305169095);
#33810=CIRCLE('',#105645,60.4792282238308);
#33811=CIRCLE('',#105646,60.4792282238308);
#33812=CIRCLE('',#105647,60.4792282238308);
#33813=CIRCLE('',#105649,60.6419265158129);
#33814=CIRCLE('',#105651,60.8618969683742);
#33815=CIRCLE('',#105652,61.0131030316259);
#33816=CIRCLE('',#105654,61.2330734841871);
#33817=CIRCLE('',#105655,61.3957717761693);
#33818=CIRCLE('',#105656,61.3957717761693);
#33819=CIRCLE('',#105657,61.3957717761693);
#33820=CIRCLE('',#105659,61.8704694830905);
#33821=CIRCLE('',#105661,0.635007073208606);
#33822=CIRCLE('',#105662,0.635007073208636);
#33823=CIRCLE('',#105673,60.0045305169095);
#33824=CIRCLE('',#105674,60.4792282238308);
#33825=CIRCLE('',#105675,60.4792282238308);
#33826=CIRCLE('',#105676,60.4792282238308);
#33827=CIRCLE('',#105678,60.6419265158129);
#33828=CIRCLE('',#105680,60.8618969683742);
#33829=CIRCLE('',#105681,61.0131030316259);
#33830=CIRCLE('',#105683,61.2330734841871);
#33831=CIRCLE('',#105684,61.3957717761693);
#33832=CIRCLE('',#105685,61.3957717761693);
#33833=CIRCLE('',#105686,61.3957717761693);
#33834=CIRCLE('',#105688,61.8704694830905);
#33835=CIRCLE('',#105690,0.635007073208653);
#33836=CIRCLE('',#105691,0.635007073208628);
#33837=CIRCLE('',#105702,60.0045305169095);
#33838=CIRCLE('',#105703,60.4792282238308);
#33839=CIRCLE('',#105704,60.4792282238308);
#33840=CIRCLE('',#105705,60.4792282238308);
#33841=CIRCLE('',#105707,60.6419265158129);
#33842=CIRCLE('',#105709,60.8618969683742);
#33843=CIRCLE('',#105710,61.0131030316259);
#33844=CIRCLE('',#105712,61.2330734841871);
#33845=CIRCLE('',#105713,61.3957717761693);
#33846=CIRCLE('',#105714,61.3957717761693);
#33847=CIRCLE('',#105715,61.3957717761693);
#33848=CIRCLE('',#105717,61.8704694830905);
#33849=CIRCLE('',#105719,0.635007073208654);
#33850=CIRCLE('',#105720,0.63500707320867);
#33851=CIRCLE('',#105731,60.0045305169095);
#33852=CIRCLE('',#105732,60.4792282238308);
#33853=CIRCLE('',#105733,60.4792282238308);
#33854=CIRCLE('',#105734,60.4792282238308);
#33855=CIRCLE('',#105736,60.6419265158129);
#33856=CIRCLE('',#105738,60.8618969683742);
#33857=CIRCLE('',#105739,61.0131030316259);
#33858=CIRCLE('',#105741,61.2330734841871);
#33859=CIRCLE('',#105742,61.3957717761693);
#33860=CIRCLE('',#105743,61.3957717761693);
#33861=CIRCLE('',#105744,61.3957717761693);
#33862=CIRCLE('',#105746,61.8704694830905);
#33863=CIRCLE('',#105748,0.635007073208616);
#33864=CIRCLE('',#105749,0.635007073208614);
#33865=CIRCLE('',#105760,60.0045305169095);
#33866=CIRCLE('',#105761,60.4792282238308);
#33867=CIRCLE('',#105762,60.4792282238308);
#33868=CIRCLE('',#105763,60.4792282238308);
#33869=CIRCLE('',#105765,60.6419265158129);
#33870=CIRCLE('',#105767,60.8618969683742);
#33871=CIRCLE('',#105768,61.0131030316259);
#33872=CIRCLE('',#105770,61.2330734841871);
#33873=CIRCLE('',#105771,61.3957717761693);
#33874=CIRCLE('',#105772,61.3957717761693);
#33875=CIRCLE('',#105773,61.3957717761693);
#33876=CIRCLE('',#105775,61.8704694830905);
#33877=CIRCLE('',#105777,0.635007073208599);
#33878=CIRCLE('',#105778,0.635007073208632);
#33879=CIRCLE('',#105789,60.0045305169095);
#33880=CIRCLE('',#105790,60.4792282238308);
#33881=CIRCLE('',#105791,60.4792282238308);
#33882=CIRCLE('',#105792,60.4792282238308);
#33883=CIRCLE('',#105794,60.6419265158129);
#33884=CIRCLE('',#105796,60.8618969683742);
#33885=CIRCLE('',#105797,61.0131030316259);
#33886=CIRCLE('',#105799,61.2330734841871);
#33887=CIRCLE('',#105800,61.3957717761693);
#33888=CIRCLE('',#105801,61.3957717761693);
#33889=CIRCLE('',#105802,61.3957717761693);
#33890=CIRCLE('',#105804,61.8704694830905);
#33891=CIRCLE('',#105806,0.635007073208614);
#33892=CIRCLE('',#105807,0.63500707320859);
#33893=CIRCLE('',#105818,60.0045305169095);
#33894=CIRCLE('',#105819,60.4792282238308);
#33895=CIRCLE('',#105820,60.4792282238308);
#33896=CIRCLE('',#105821,60.4792282238308);
#33897=CIRCLE('',#105823,60.6419265158129);
#33898=CIRCLE('',#105825,60.8618969683742);
#33899=CIRCLE('',#105826,61.0131030316259);
#33900=CIRCLE('',#105828,61.2330734841871);
#33901=CIRCLE('',#105829,61.3957717761693);
#33902=CIRCLE('',#105830,61.3957717761693);
#33903=CIRCLE('',#105831,61.3957717761693);
#33904=CIRCLE('',#105833,61.8704694830905);
#33905=CIRCLE('',#105835,0.635007073208637);
#33906=CIRCLE('',#105836,0.635007073208625);
#33907=CIRCLE('',#105847,60.0045305169095);
#33908=CIRCLE('',#105848,60.4792282238308);
#33909=CIRCLE('',#105849,60.4792282238308);
#33910=CIRCLE('',#105850,60.4792282238308);
#33911=CIRCLE('',#105852,60.6419265158129);
#33912=CIRCLE('',#105854,60.8618969683742);
#33913=CIRCLE('',#105855,61.0131030316259);
#33914=CIRCLE('',#105857,61.2330734841871);
#33915=CIRCLE('',#105858,61.3957717761693);
#33916=CIRCLE('',#105859,61.3957717761693);
#33917=CIRCLE('',#105860,61.3957717761693);
#33918=CIRCLE('',#105862,61.8704694830905);
#33919=CIRCLE('',#105864,0.635007073208638);
#33920=CIRCLE('',#105865,0.635007073208649);
#33921=CIRCLE('',#105876,60.0045305169095);
#33922=CIRCLE('',#105877,60.4792282238308);
#33923=CIRCLE('',#105878,60.4792282238308);
#33924=CIRCLE('',#105879,60.4792282238308);
#33925=CIRCLE('',#105881,60.6419265158129);
#33926=CIRCLE('',#105883,60.8618969683742);
#33927=CIRCLE('',#105884,61.0131030316259);
#33928=CIRCLE('',#105886,61.2330734841871);
#33929=CIRCLE('',#105887,61.3957717761693);
#33930=CIRCLE('',#105888,61.3957717761693);
#33931=CIRCLE('',#105889,61.3957717761693);
#33932=CIRCLE('',#105891,61.8704694830905);
#33933=CIRCLE('',#105893,0.635007073208641);
#33934=CIRCLE('',#105894,0.635007073208602);
#33935=CIRCLE('',#105905,60.0045305169095);
#33936=CIRCLE('',#105906,60.4792282238308);
#33937=CIRCLE('',#105907,60.4792282238308);
#33938=CIRCLE('',#105908,60.4792282238308);
#33939=CIRCLE('',#105910,60.6419265158129);
#33940=CIRCLE('',#105912,60.8618969683742);
#33941=CIRCLE('',#105913,61.0131030316259);
#33942=CIRCLE('',#105915,61.2330734841871);
#33943=CIRCLE('',#105916,61.3957717761693);
#33944=CIRCLE('',#105917,61.3957717761693);
#33945=CIRCLE('',#105918,61.3957717761693);
#33946=CIRCLE('',#105920,61.8704694830905);
#33947=CIRCLE('',#105922,0.635007073208628);
#33948=CIRCLE('',#105923,0.635007073208635);
#33949=CIRCLE('',#105934,60.0045305169095);
#33950=CIRCLE('',#105935,60.4792282238308);
#33951=CIRCLE('',#105936,60.4792282238308);
#33952=CIRCLE('',#105937,60.4792282238308);
#33953=CIRCLE('',#105939,60.6419265158129);
#33954=CIRCLE('',#105941,60.8618969683742);
#33955=CIRCLE('',#105942,61.0131030316259);
#33956=CIRCLE('',#105944,61.2330734841871);
#33957=CIRCLE('',#105945,61.3957717761693);
#33958=CIRCLE('',#105946,61.3957717761693);
#33959=CIRCLE('',#105947,61.3957717761693);
#33960=CIRCLE('',#105949,61.8704694830905);
#33961=CIRCLE('',#105951,0.63500707320863);
#33962=CIRCLE('',#105952,0.635007073208594);
#33963=CIRCLE('',#105963,60.0045305169095);
#33964=CIRCLE('',#105964,60.4792282238308);
#33965=CIRCLE('',#105965,60.4792282238308);
#33966=CIRCLE('',#105966,60.4792282238308);
#33967=CIRCLE('',#105968,60.6419265158129);
#33968=CIRCLE('',#105970,60.8618969683742);
#33969=CIRCLE('',#105971,61.0131030316259);
#33970=CIRCLE('',#105973,61.2330734841871);
#33971=CIRCLE('',#105974,61.3957717761693);
#33972=CIRCLE('',#105975,61.3957717761693);
#33973=CIRCLE('',#105976,61.3957717761693);
#33974=CIRCLE('',#105978,61.8704694830905);
#33975=CIRCLE('',#105980,0.635007073208599);
#33976=CIRCLE('',#105981,0.635007073208596);
#33977=CIRCLE('',#105992,60.0045305169095);
#33978=CIRCLE('',#105993,60.4792282238308);
#33979=CIRCLE('',#105994,60.4792282238308);
#33980=CIRCLE('',#105995,60.4792282238308);
#33981=CIRCLE('',#105997,60.6419265158129);
#33982=CIRCLE('',#105999,60.8618969683742);
#33983=CIRCLE('',#106000,61.0131030316259);
#33984=CIRCLE('',#106002,61.2330734841871);
#33985=CIRCLE('',#106003,61.3957717761693);
#33986=CIRCLE('',#106004,61.3957717761693);
#33987=CIRCLE('',#106005,61.3957717761693);
#33988=CIRCLE('',#106007,61.8704694830905);
#33989=CIRCLE('',#106009,0.635007073208624);
#33990=CIRCLE('',#106010,0.635007073208611);
#33991=CIRCLE('',#106021,60.0045305169095);
#33992=CIRCLE('',#106022,60.4792282238308);
#33993=CIRCLE('',#106023,60.4792282238308);
#33994=CIRCLE('',#106024,60.4792282238308);
#33995=CIRCLE('',#106026,60.6419265158129);
#33996=CIRCLE('',#106028,60.8618969683742);
#33997=CIRCLE('',#106029,61.0131030316259);
#33998=CIRCLE('',#106031,61.2330734841871);
#33999=CIRCLE('',#106032,61.3957717761693);
#34000=CIRCLE('',#106033,61.3957717761693);
#34001=CIRCLE('',#106034,61.3957717761693);
#34002=CIRCLE('',#106036,61.8704694830905);
#34003=CIRCLE('',#106038,0.635007073208621);
#34004=CIRCLE('',#106039,0.6350070732086);
#34005=CIRCLE('',#106050,60.0045305169095);
#34006=CIRCLE('',#106051,60.4792282238308);
#34007=CIRCLE('',#106052,60.4792282238308);
#34008=CIRCLE('',#106053,60.4792282238308);
#34009=CIRCLE('',#106055,60.6419265158129);
#34010=CIRCLE('',#106057,60.8618969683742);
#34011=CIRCLE('',#106058,61.0131030316259);
#34012=CIRCLE('',#106060,61.2330734841871);
#34013=CIRCLE('',#106061,61.3957717761693);
#34014=CIRCLE('',#106062,61.3957717761693);
#34015=CIRCLE('',#106063,61.3957717761693);
#34016=CIRCLE('',#106065,61.8704694830905);
#34017=CIRCLE('',#106067,0.635007073208618);
#34018=CIRCLE('',#106068,0.635007073208615);
#34019=CIRCLE('',#106079,60.0045305169095);
#34020=CIRCLE('',#106080,60.4792282238308);
#34021=CIRCLE('',#106081,60.4792282238308);
#34022=CIRCLE('',#106082,60.4792282238308);
#34023=CIRCLE('',#106084,60.6419265158129);
#34024=CIRCLE('',#106086,60.8618969683742);
#34025=CIRCLE('',#106087,61.0131030316259);
#34026=CIRCLE('',#106089,61.2330734841871);
#34027=CIRCLE('',#106090,61.3957717761693);
#34028=CIRCLE('',#106091,61.3957717761693);
#34029=CIRCLE('',#106092,61.3957717761693);
#34030=CIRCLE('',#106094,61.8704694830905);
#34031=CIRCLE('',#106096,0.635007073208615);
#34032=CIRCLE('',#106097,0.6350070732086);
#34033=CIRCLE('',#106108,60.0045305169095);
#34034=CIRCLE('',#106109,60.4792282238308);
#34035=CIRCLE('',#106110,60.4792282238308);
#34036=CIRCLE('',#106111,60.4792282238308);
#34037=CIRCLE('',#106113,60.6419265158129);
#34038=CIRCLE('',#106115,60.8618969683742);
#34039=CIRCLE('',#106116,61.0131030316259);
#34040=CIRCLE('',#106118,61.2330734841871);
#34041=CIRCLE('',#106119,61.3957717761693);
#34042=CIRCLE('',#106120,61.3957717761693);
#34043=CIRCLE('',#106121,61.3957717761693);
#34044=CIRCLE('',#106123,61.8704694830905);
#34045=CIRCLE('',#106125,0.635007073208631);
#34046=CIRCLE('',#106126,0.635007073208609);
#34047=CIRCLE('',#106137,60.0045305169095);
#34048=CIRCLE('',#106138,60.4792282238308);
#34049=CIRCLE('',#106139,60.4792282238308);
#34050=CIRCLE('',#106140,60.4792282238308);
#34051=CIRCLE('',#106142,60.6419265158129);
#34052=CIRCLE('',#106144,60.8618969683742);
#34053=CIRCLE('',#106145,61.0131030316259);
#34054=CIRCLE('',#106147,61.2330734841871);
#34055=CIRCLE('',#106148,61.3957717761693);
#34056=CIRCLE('',#106149,61.3957717761693);
#34057=CIRCLE('',#106150,61.3957717761693);
#34058=CIRCLE('',#106152,61.8704694830905);
#34059=CIRCLE('',#106154,0.635007073208616);
#34060=CIRCLE('',#106155,0.635007073208572);
#34061=CIRCLE('',#106166,60.0045305169095);
#34062=CIRCLE('',#106167,60.4792282238308);
#34063=CIRCLE('',#106168,60.4792282238308);
#34064=CIRCLE('',#106169,60.4792282238308);
#34065=CIRCLE('',#106171,60.6419265158129);
#34066=CIRCLE('',#106173,60.8618969683742);
#34067=CIRCLE('',#106174,61.0131030316259);
#34068=CIRCLE('',#106176,61.2330734841871);
#34069=CIRCLE('',#106177,61.3957717761693);
#34070=CIRCLE('',#106178,61.3957717761693);
#34071=CIRCLE('',#106179,61.3957717761693);
#34072=CIRCLE('',#106181,61.8704694830905);
#34073=CIRCLE('',#106183,0.635007073208599);
#34074=CIRCLE('',#106184,0.635007073208599);
#34075=CIRCLE('',#106195,60.0045305169095);
#34076=CIRCLE('',#106196,60.4792282238308);
#34077=CIRCLE('',#106197,60.4792282238308);
#34078=CIRCLE('',#106198,60.4792282238308);
#34079=CIRCLE('',#106200,60.6419265158129);
#34080=CIRCLE('',#106202,60.8618969683742);
#34081=CIRCLE('',#106203,61.0131030316259);
#34082=CIRCLE('',#106205,61.2330734841871);
#34083=CIRCLE('',#106206,61.3957717761693);
#34084=CIRCLE('',#106207,61.3957717761693);
#34085=CIRCLE('',#106208,61.3957717761693);
#34086=CIRCLE('',#106210,61.8704694830905);
#34087=CIRCLE('',#106212,0.635007073208628);
#34088=CIRCLE('',#106213,0.635007073208624);
#34089=CIRCLE('',#106224,60.0045305169095);
#34090=CIRCLE('',#106225,60.4792282238308);
#34091=CIRCLE('',#106226,60.4792282238308);
#34092=CIRCLE('',#106227,60.4792282238308);
#34093=CIRCLE('',#106229,60.6419265158129);
#34094=CIRCLE('',#106231,60.8618969683742);
#34095=CIRCLE('',#106232,61.0131030316259);
#34096=CIRCLE('',#106234,61.2330734841871);
#34097=CIRCLE('',#106235,61.3957717761693);
#34098=CIRCLE('',#106236,61.3957717761693);
#34099=CIRCLE('',#106237,61.3957717761693);
#34100=CIRCLE('',#106239,61.8704694830905);
#34101=CIRCLE('',#106241,0.635007073208624);
#34102=CIRCLE('',#106242,0.635007073208604);
#34103=CIRCLE('',#106253,60.0045305169095);
#34104=CIRCLE('',#106254,60.4792282238308);
#34105=CIRCLE('',#106255,60.4792282238308);
#34106=CIRCLE('',#106256,60.4792282238308);
#34107=CIRCLE('',#106258,60.6419265158129);
#34108=CIRCLE('',#106260,60.8618969683742);
#34109=CIRCLE('',#106261,61.0131030316259);
#34110=CIRCLE('',#106263,61.2330734841871);
#34111=CIRCLE('',#106264,61.3957717761693);
#34112=CIRCLE('',#106265,61.3957717761693);
#34113=CIRCLE('',#106266,61.3957717761693);
#34114=CIRCLE('',#106268,61.8704694830905);
#34115=CIRCLE('',#106270,0.635007073208647);
#34116=CIRCLE('',#106271,0.635007073208648);
#34117=CIRCLE('',#106282,60.0045305169095);
#34118=CIRCLE('',#106283,60.4792282238308);
#34119=CIRCLE('',#106284,60.4792282238308);
#34120=CIRCLE('',#106285,60.4792282238308);
#34121=CIRCLE('',#106287,60.6419265158129);
#34122=CIRCLE('',#106289,60.8618969683742);
#34123=CIRCLE('',#106290,61.0131030316259);
#34124=CIRCLE('',#106292,61.2330734841871);
#34125=CIRCLE('',#106293,61.3957717761693);
#34126=CIRCLE('',#106294,61.3957717761693);
#34127=CIRCLE('',#106295,61.3957717761693);
#34128=CIRCLE('',#106297,61.8704694830905);
#34129=CIRCLE('',#106299,0.63500707320862);
#34130=CIRCLE('',#106300,0.635007073208608);
#34131=CIRCLE('',#106311,60.0045305169095);
#34132=CIRCLE('',#106312,60.4792282238308);
#34133=CIRCLE('',#106313,60.4792282238308);
#34134=CIRCLE('',#106314,60.4792282238308);
#34135=CIRCLE('',#106316,60.6419265158129);
#34136=CIRCLE('',#106318,60.8618969683742);
#34137=CIRCLE('',#106319,61.0131030316259);
#34138=CIRCLE('',#106321,61.2330734841871);
#34139=CIRCLE('',#106322,61.3957717761693);
#34140=CIRCLE('',#106323,61.3957717761693);
#34141=CIRCLE('',#106324,61.3957717761693);
#34142=CIRCLE('',#106326,61.8704694830905);
#34143=CIRCLE('',#106328,0.635007073208603);
#34144=CIRCLE('',#106329,0.635007073208596);
#34145=CIRCLE('',#106340,60.0045305169095);
#34146=CIRCLE('',#106341,60.4792282238308);
#34147=CIRCLE('',#106342,60.4792282238308);
#34148=CIRCLE('',#106343,60.4792282238308);
#34149=CIRCLE('',#106345,60.6419265158129);
#34150=CIRCLE('',#106347,60.8618969683742);
#34151=CIRCLE('',#106348,61.0131030316259);
#34152=CIRCLE('',#106350,61.2330734841871);
#34153=CIRCLE('',#106351,61.3957717761693);
#34154=CIRCLE('',#106352,61.3957717761693);
#34155=CIRCLE('',#106353,61.3957717761693);
#34156=CIRCLE('',#106355,61.8704694830905);
#34157=CIRCLE('',#106357,0.635007073208654);
#34158=CIRCLE('',#106358,0.6350070732086);
#34159=CIRCLE('',#106369,60.0045305169095);
#34160=CIRCLE('',#106370,60.4792282238308);
#34161=CIRCLE('',#106371,60.4792282238308);
#34162=CIRCLE('',#106372,60.4792282238308);
#34163=CIRCLE('',#106374,60.6419265158129);
#34164=CIRCLE('',#106376,60.8618969683742);
#34165=CIRCLE('',#106377,61.0131030316259);
#34166=CIRCLE('',#106379,61.2330734841871);
#34167=CIRCLE('',#106380,61.3957717761693);
#34168=CIRCLE('',#106381,61.3957717761693);
#34169=CIRCLE('',#106382,61.3957717761693);
#34170=CIRCLE('',#106384,61.8704694830905);
#34171=CIRCLE('',#106386,0.635007073208615);
#34172=CIRCLE('',#106387,0.635007073208638);
#34173=CIRCLE('',#106398,60.0045305169095);
#34174=CIRCLE('',#106399,60.4792282238308);
#34175=CIRCLE('',#106400,60.4792282238308);
#34176=CIRCLE('',#106401,60.4792282238308);
#34177=CIRCLE('',#106403,60.6419265158129);
#34178=CIRCLE('',#106405,60.8618969683742);
#34179=CIRCLE('',#106406,61.0131030316259);
#34180=CIRCLE('',#106408,61.2330734841871);
#34181=CIRCLE('',#106409,61.3957717761693);
#34182=CIRCLE('',#106410,61.3957717761693);
#34183=CIRCLE('',#106411,61.3957717761693);
#34184=CIRCLE('',#106413,61.8704694830905);
#34185=CIRCLE('',#106415,0.635007073208598);
#34186=CIRCLE('',#106416,0.635007073208636);
#34187=CIRCLE('',#106427,60.0045305169095);
#34188=CIRCLE('',#106428,60.4792282238308);
#34189=CIRCLE('',#106429,60.4792282238308);
#34190=CIRCLE('',#106430,60.4792282238308);
#34191=CIRCLE('',#106432,60.6419265158129);
#34192=CIRCLE('',#106434,60.8618969683742);
#34193=CIRCLE('',#106435,61.0131030316259);
#34194=CIRCLE('',#106437,61.2330734841871);
#34195=CIRCLE('',#106438,61.3957717761693);
#34196=CIRCLE('',#106439,61.3957717761693);
#34197=CIRCLE('',#106440,61.3957717761693);
#34198=CIRCLE('',#106442,61.8704694830905);
#34199=CIRCLE('',#106444,0.635007073208679);
#34200=CIRCLE('',#106445,0.635007073208629);
#34201=CIRCLE('',#106456,60.0045305169095);
#34202=CIRCLE('',#106457,60.4792282238308);
#34203=CIRCLE('',#106458,60.4792282238308);
#34204=CIRCLE('',#106459,60.4792282238308);
#34205=CIRCLE('',#106461,60.6419265158129);
#34206=CIRCLE('',#106463,60.8618969683742);
#34207=CIRCLE('',#106464,61.0131030316259);
#34208=CIRCLE('',#106466,61.2330734841871);
#34209=CIRCLE('',#106467,61.3957717761693);
#34210=CIRCLE('',#106468,61.3957717761693);
#34211=CIRCLE('',#106469,61.3957717761693);
#34212=CIRCLE('',#106471,61.8704694830905);
#34213=CIRCLE('',#106473,0.63500707320862);
#34214=CIRCLE('',#106474,0.635007073208651);
#34215=CIRCLE('',#106485,60.0045305169095);
#34216=CIRCLE('',#106486,60.4792282238308);
#34217=CIRCLE('',#106487,60.4792282238308);
#34218=CIRCLE('',#106488,60.4792282238308);
#34219=CIRCLE('',#106490,60.6419265158129);
#34220=CIRCLE('',#106492,60.8618969683742);
#34221=CIRCLE('',#106493,61.0131030316259);
#34222=CIRCLE('',#106495,61.2330734841871);
#34223=CIRCLE('',#106496,61.3957717761693);
#34224=CIRCLE('',#106497,61.3957717761693);
#34225=CIRCLE('',#106498,61.3957717761693);
#34226=CIRCLE('',#106500,61.8704694830905);
#34227=CIRCLE('',#106502,0.635007073208615);
#34228=CIRCLE('',#106503,0.635007073208618);
#34229=CIRCLE('',#106514,60.0045305169095);
#34230=CIRCLE('',#106515,60.4792282238308);
#34231=CIRCLE('',#106516,60.4792282238308);
#34232=CIRCLE('',#106517,60.4792282238308);
#34233=CIRCLE('',#106519,60.6419265158129);
#34234=CIRCLE('',#106521,60.8618969683742);
#34235=CIRCLE('',#106522,61.0131030316259);
#34236=CIRCLE('',#106524,61.2330734841871);
#34237=CIRCLE('',#106525,61.3957717761693);
#34238=CIRCLE('',#106526,61.3957717761693);
#34239=CIRCLE('',#106527,61.3957717761693);
#34240=CIRCLE('',#106529,61.8704694830905);
#34241=CIRCLE('',#106531,0.635007073208631);
#34242=CIRCLE('',#106532,0.63500707320861);
#34243=CIRCLE('',#106543,60.0045305169095);
#34244=CIRCLE('',#106544,60.4792282238308);
#34245=CIRCLE('',#106545,60.4792282238308);
#34246=CIRCLE('',#106546,60.4792282238308);
#34247=CIRCLE('',#106548,60.6419265158129);
#34248=CIRCLE('',#106550,60.8618969683742);
#34249=CIRCLE('',#106551,61.0131030316259);
#34250=CIRCLE('',#106553,61.2330734841871);
#34251=CIRCLE('',#106554,61.3957717761693);
#34252=CIRCLE('',#106555,61.3957717761693);
#34253=CIRCLE('',#106556,61.3957717761693);
#34254=CIRCLE('',#106558,61.8704694830905);
#34255=CIRCLE('',#106560,0.635007073208622);
#34256=CIRCLE('',#106561,0.635007073208639);
#34257=CIRCLE('',#106572,60.0045305169095);
#34258=CIRCLE('',#106573,60.4792282238308);
#34259=CIRCLE('',#106574,60.4792282238308);
#34260=CIRCLE('',#106575,60.4792282238308);
#34261=CIRCLE('',#106577,60.6419265158129);
#34262=CIRCLE('',#106579,60.8618969683742);
#34263=CIRCLE('',#106580,61.0131030316259);
#34264=CIRCLE('',#106582,61.2330734841871);
#34265=CIRCLE('',#106583,61.3957717761693);
#34266=CIRCLE('',#106584,61.3957717761693);
#34267=CIRCLE('',#106585,61.3957717761693);
#34268=CIRCLE('',#106587,61.8704694830905);
#34269=CIRCLE('',#106589,0.635007073208608);
#34270=CIRCLE('',#106590,0.635007073208623);
#34271=CIRCLE('',#106601,60.0045305169095);
#34272=CIRCLE('',#106602,60.4792282238308);
#34273=CIRCLE('',#106603,60.4792282238308);
#34274=CIRCLE('',#106604,60.4792282238308);
#34275=CIRCLE('',#106606,60.6419265158129);
#34276=CIRCLE('',#106608,60.8618969683742);
#34277=CIRCLE('',#106609,61.0131030316259);
#34278=CIRCLE('',#106611,61.2330734841871);
#34279=CIRCLE('',#106612,61.3957717761693);
#34280=CIRCLE('',#106613,61.3957717761693);
#34281=CIRCLE('',#106614,61.3957717761693);
#34282=CIRCLE('',#106616,61.8704694830905);
#34283=CIRCLE('',#106618,0.635007073208607);
#34284=CIRCLE('',#106619,0.635007073208629);
#34285=CIRCLE('',#106631,60.0045305169095);
#34286=CIRCLE('',#106632,60.4792282238308);
#34287=CIRCLE('',#106633,60.4792282238308);
#34288=CIRCLE('',#106634,60.4792282238308);
#34289=CIRCLE('',#106636,60.6419265158129);
#34290=CIRCLE('',#106638,60.8618969683742);
#34291=CIRCLE('',#106639,61.0131030316259);
#34292=CIRCLE('',#106641,61.2330734841871);
#34293=CIRCLE('',#106642,61.3957717761693);
#34294=CIRCLE('',#106643,61.3957717761693);
#34295=CIRCLE('',#106644,61.3957717761693);
#34296=CIRCLE('',#106646,61.8704694830905);
#34297=CIRCLE('',#106650,0.635007073208622);
#34298=CIRCLE('',#106651,0.635007073208615);
#34299=CIRCLE('',#106662,62.8464445485378);
#34300=CIRCLE('',#106663,59.0285554514622);
#34301=CIRCLE('',#106678,0.127);
#34302=CIRCLE('',#106679,0.127);
#34303=CIRCLE('',#106681,0.127);
#34304=CIRCLE('',#106683,0.127);
#34305=CIRCLE('',#106684,0.126999999999997);
#34306=CIRCLE('',#106685,0.127000000000002);
#34307=CIRCLE('',#106687,0.127000000000005);
#34308=CIRCLE('',#106690,0.127000000000002);
#34309=CIRCLE('',#106692,0.127);
#34310=CIRCLE('',#106694,0.127000000000002);
#34311=CIRCLE('',#106695,0.127);
#34312=CIRCLE('',#106696,0.127000000000005);
#34313=CIRCLE('',#106698,0.126999999999998);
#34314=CIRCLE('',#106700,0.126999999999999);
#34315=CIRCLE('',#106701,0.127000000000002);
#34316=CIRCLE('',#106702,0.127);
#34317=CIRCLE('',#106704,0.127000000000002);
#34318=CIRCLE('',#106707,0.126999999999998);
#34319=CIRCLE('',#106709,0.127);
#34320=CIRCLE('',#106711,0.127);
#34321=CIRCLE('',#106712,0.127);
#34322=CIRCLE('',#106713,0.127);
#34323=CIRCLE('',#106715,0.127);
#34324=CIRCLE('',#106718,0.127);
#34325=CIRCLE('',#106721,62.8464445485378);
#34326=CIRCLE('',#106722,59.0285554514622);
#34327=CIRCLE('',#106734,62.8464445485378);
#34328=CIRCLE('',#106735,59.0285554514622);
#34329=CIRCLE('',#106747,62.8464445485378);
#34330=CIRCLE('',#106748,59.0285554514622);
#34331=CIRCLE('',#106760,62.8464445485378);
#34332=CIRCLE('',#106761,59.0285554514622);
#34333=CIRCLE('',#106773,62.8464445485378);
#34334=CIRCLE('',#106774,59.0285554514622);
#34335=CIRCLE('',#106786,62.8464445485378);
#34336=CIRCLE('',#106787,59.0285554514622);
#34337=CIRCLE('',#106799,62.8464445485378);
#34338=CIRCLE('',#106800,59.0285554514622);
#34339=CIRCLE('',#106812,62.8464445485378);
#34340=CIRCLE('',#106813,59.0285554514622);
#34341=CIRCLE('',#106825,62.8464445485378);
#34342=CIRCLE('',#106826,59.0285554514622);
#34343=CIRCLE('',#106838,62.8464445485378);
#34344=CIRCLE('',#106839,59.0285554514622);
#34345=CIRCLE('',#106851,62.8464445485378);
#34346=CIRCLE('',#106852,59.0285554514622);
#34347=CIRCLE('',#106864,62.8464445485378);
#34348=CIRCLE('',#106865,59.0285554514622);
#34349=CIRCLE('',#106877,62.8464445485378);
#34350=CIRCLE('',#106878,59.0285554514622);
#34351=CIRCLE('',#106890,62.8464445485378);
#34352=CIRCLE('',#106891,59.0285554514622);
#34353=CIRCLE('',#106903,62.8464445485378);
#34354=CIRCLE('',#106904,59.0285554514622);
#34355=CIRCLE('',#106916,62.8464445485378);
#34356=CIRCLE('',#106917,59.0285554514622);
#34357=CIRCLE('',#106929,62.8464445485378);
#34358=CIRCLE('',#106930,59.0285554514622);
#34359=CIRCLE('',#106942,62.8464445485378);
#34360=CIRCLE('',#106943,59.0285554514622);
#34361=CIRCLE('',#106955,62.8464445485378);
#34362=CIRCLE('',#106956,59.0285554514622);
#34363=CIRCLE('',#106968,62.8464445485378);
#34364=CIRCLE('',#106969,59.0285554514622);
#34365=CIRCLE('',#106981,62.8464445485378);
#34366=CIRCLE('',#106982,59.0285554514622);
#34367=CIRCLE('',#106994,62.8464445485378);
#34368=CIRCLE('',#106995,59.0285554514622);
#34369=CIRCLE('',#107007,62.8464445485378);
#34370=CIRCLE('',#107008,59.0285554514622);
#34371=CIRCLE('',#107020,62.8464445485378);
#34372=CIRCLE('',#107021,59.0285554514622);
#34373=CIRCLE('',#107033,62.8464445485378);
#34374=CIRCLE('',#107034,59.0285554514622);
#34375=CIRCLE('',#107046,62.8464445485378);
#34376=CIRCLE('',#107047,59.0285554514622);
#34377=CIRCLE('',#107059,62.8464445485378);
#34378=CIRCLE('',#107060,59.0285554514622);
#34379=CIRCLE('',#107072,62.8464445485378);
#34380=CIRCLE('',#107073,59.0285554514622);
#34381=CIRCLE('',#107085,62.8464445485378);
#34382=CIRCLE('',#107086,59.0285554514622);
#34383=CIRCLE('',#107109,62.8464445485378);
#34384=CIRCLE('',#107110,59.0285554514622);
#34385=CIRCLE('',#107122,62.8464445485378);
#34386=CIRCLE('',#107123,59.0285554514622);
#34387=CIRCLE('',#107135,62.8464445485378);
#34388=CIRCLE('',#107136,59.0285554514622);
#34389=CIRCLE('',#107148,62.8464445485378);
#34390=CIRCLE('',#107149,59.0285554514622);
#34391=CIRCLE('',#107161,62.8464445485378);
#34392=CIRCLE('',#107162,59.0285554514622);
#34393=CIRCLE('',#107174,62.8464445485378);
#34394=CIRCLE('',#107175,59.0285554514622);
#34395=CIRCLE('',#107187,62.8464445485378);
#34396=CIRCLE('',#107188,59.0285554514622);
#34397=CIRCLE('',#107200,62.8464445485378);
#34398=CIRCLE('',#107201,59.0285554514622);
#34399=CIRCLE('',#107213,62.8464445485378);
#34400=CIRCLE('',#107214,59.0285554514622);
#34401=CIRCLE('',#107226,62.8464445485378);
#34402=CIRCLE('',#107227,59.0285554514622);
#34403=CIRCLE('',#107239,62.8464445485378);
#34404=CIRCLE('',#107240,59.0285554514622);
#34405=CIRCLE('',#107252,62.8464445485378);
#34406=CIRCLE('',#107253,59.0285554514622);
#34407=CIRCLE('',#107265,62.8464445485378);
#34408=CIRCLE('',#107266,59.0285554514622);
#34409=CIRCLE('',#107278,62.8464445485378);
#34410=CIRCLE('',#107279,59.0285554514622);
#34411=CIRCLE('',#107302,62.8464445485378);
#34412=CIRCLE('',#107303,59.0285554514622);
#34413=CIRCLE('',#107315,62.8464445485378);
#34414=CIRCLE('',#107316,59.0285554514622);
#34415=CIRCLE('',#107328,62.8464445485378);
#34416=CIRCLE('',#107329,59.0285554514622);
#34417=CIRCLE('',#107341,62.8464445485378);
#34418=CIRCLE('',#107342,59.0285554514622);
#34419=CIRCLE('',#107354,62.8464445485378);
#34420=CIRCLE('',#107355,59.0285554514622);
#34421=CIRCLE('',#107367,62.8464445485378);
#34422=CIRCLE('',#107368,59.0285554514622);
#34423=CIRCLE('',#107380,62.8464445485378);
#34424=CIRCLE('',#107381,59.0285554514622);
#34425=CIRCLE('',#107393,62.8464445485378);
#34426=CIRCLE('',#107394,59.0285554514622);
#34427=CIRCLE('',#107406,62.8464445485378);
#34428=CIRCLE('',#107407,59.0285554514622);
#34429=CIRCLE('',#107419,62.8464445485378);
#34430=CIRCLE('',#107420,59.0285554514622);
#34431=CIRCLE('',#107432,62.8464445485378);
#34432=CIRCLE('',#107433,59.0285554514622);
#34433=CIRCLE('',#107445,62.8464445485378);
#34434=CIRCLE('',#107446,59.0285554514622);
#34435=CIRCLE('',#107458,62.8464445485378);
#34436=CIRCLE('',#107459,59.0285554514622);
#34437=CIRCLE('',#107471,62.8464445485378);
#34438=CIRCLE('',#107472,59.0285554514622);
#34439=CIRCLE('',#107603,0.126999999999997);
#34440=CIRCLE('',#107604,0.127);
#34441=CIRCLE('',#107606,0.127);
#34442=CIRCLE('',#107608,0.127);
#34443=CIRCLE('',#107609,0.127000000000001);
#34444=CIRCLE('',#107610,0.127000000000001);
#34445=CIRCLE('',#107612,0.127);
#34446=CIRCLE('',#107615,0.127000000000004);
#34447=CIRCLE('',#107617,0.127);
#34448=CIRCLE('',#107619,0.127000000000002);
#34449=CIRCLE('',#107620,0.127000000000001);
#34450=CIRCLE('',#107621,0.126999999999998);
#34451=CIRCLE('',#107623,0.127);
#34452=CIRCLE('',#107625,0.127000000000002);
#34453=CIRCLE('',#107626,0.127);
#34454=CIRCLE('',#107627,0.127);
#34455=CIRCLE('',#107629,0.126999999999997);
#34456=CIRCLE('',#107632,0.127);
#34457=CIRCLE('',#107634,0.127000000000002);
#34458=CIRCLE('',#107636,0.127000000000003);
#34459=CIRCLE('',#107637,0.127);
#34460=CIRCLE('',#107638,0.127);
#34461=CIRCLE('',#107640,0.127);
#34462=CIRCLE('',#107643,0.127);
#34463=CIRCLE('',#107647,0.127);
#34464=CIRCLE('',#107648,0.126999999999999);
#34465=CIRCLE('',#107650,0.126999999999999);
#34466=CIRCLE('',#107652,0.126999999999999);
#34467=CIRCLE('',#107653,0.127000000000002);
#34468=CIRCLE('',#107654,0.127000000000003);
#34469=CIRCLE('',#107656,0.127000000000001);
#34470=CIRCLE('',#107659,0.127000000000003);
#34471=CIRCLE('',#107661,0.126999999999999);
#34472=CIRCLE('',#107663,0.126999999999997);
#34473=CIRCLE('',#107664,0.127);
#34474=CIRCLE('',#107665,0.127000000000002);
#34475=CIRCLE('',#107667,0.127000000000003);
#34476=CIRCLE('',#107669,0.126999999999999);
#34477=CIRCLE('',#107670,0.127000000000002);
#34478=CIRCLE('',#107671,0.126999999999999);
#34479=CIRCLE('',#107673,0.127000000000001);
#34480=CIRCLE('',#107676,0.127000000000003);
#34481=CIRCLE('',#107678,0.126999999999999);
#34482=CIRCLE('',#107680,0.127000000000002);
#34483=CIRCLE('',#107681,0.126999999999999);
#34484=CIRCLE('',#107682,0.126999999999999);
#34485=CIRCLE('',#107684,0.126999999999999);
#34486=CIRCLE('',#107687,0.127000000000001);
#34487=CIRCLE('',#107691,0.127000000000003);
#34488=CIRCLE('',#107692,0.126999999999999);
#34489=CIRCLE('',#107694,0.126999999999999);
#34490=CIRCLE('',#107696,0.127);
#34491=CIRCLE('',#107697,0.127);
#34492=CIRCLE('',#107698,0.126999999999998);
#34493=CIRCLE('',#107700,0.126999999999998);
#34494=CIRCLE('',#107703,0.126999999999997);
#34495=CIRCLE('',#107705,0.127);
#34496=CIRCLE('',#107707,0.127000000000001);
#34497=CIRCLE('',#107708,0.127000000000002);
#34498=CIRCLE('',#107709,0.127000000000002);
#34499=CIRCLE('',#107711,0.126999999999997);
#34500=CIRCLE('',#107713,0.127000000000002);
#34501=CIRCLE('',#107714,0.127000000000003);
#34502=CIRCLE('',#107715,0.126999999999999);
#34503=CIRCLE('',#107717,0.127);
#34504=CIRCLE('',#107720,0.126999999999997);
#34505=CIRCLE('',#107722,0.127);
#34506=CIRCLE('',#107724,0.127);
#34507=CIRCLE('',#107725,0.126999999999999);
#34508=CIRCLE('',#107726,0.126999999999999);
#34509=CIRCLE('',#107728,0.126999999999999);
#34510=CIRCLE('',#107731,0.127000000000002);
#34511=CIRCLE('',#107735,0.126999999999998);
#34512=CIRCLE('',#107736,0.127000000000001);
#34513=CIRCLE('',#107738,0.127000000000001);
#34514=CIRCLE('',#107740,0.127000000000001);
#34515=CIRCLE('',#107741,0.127);
#34516=CIRCLE('',#107742,0.127000000000001);
#34517=CIRCLE('',#107744,0.127);
#34518=CIRCLE('',#107747,0.127000000000002);
#34519=CIRCLE('',#107749,0.127000000000001);
#34520=CIRCLE('',#107751,0.127000000000001);
#34521=CIRCLE('',#107752,0.126999999999998);
#34522=CIRCLE('',#107753,0.127);
#34523=CIRCLE('',#107755,0.126999999999999);
#34524=CIRCLE('',#107757,0.127000000000002);
#34525=CIRCLE('',#107758,0.127000000000002);
#34526=CIRCLE('',#107759,0.127000000000001);
#34527=CIRCLE('',#107761,0.126999999999997);
#34528=CIRCLE('',#107764,0.126999999999999);
#34529=CIRCLE('',#107766,0.126999999999998);
#34530=CIRCLE('',#107768,0.126999999999998);
#34531=CIRCLE('',#107769,0.127000000000001);
#34532=CIRCLE('',#107770,0.127000000000001);
#34533=CIRCLE('',#107772,0.127000000000001);
#34534=CIRCLE('',#107775,0.127000000000002);
#34535=CIRCLE('',#107779,0.127000000000001);
#34536=CIRCLE('',#107780,0.127);
#34537=CIRCLE('',#107782,0.127000000000003);
#34538=CIRCLE('',#107784,0.127);
#34539=CIRCLE('',#107785,0.126999999999998);
#34540=CIRCLE('',#107786,0.126999999999999);
#34541=CIRCLE('',#107788,0.127);
#34542=CIRCLE('',#107791,0.127000000000002);
#34543=CIRCLE('',#107793,0.127);
#34544=CIRCLE('',#107795,0.127000000000002);
#34545=CIRCLE('',#107796,0.127000000000002);
#34546=CIRCLE('',#107797,0.127);
#34547=CIRCLE('',#107799,0.127000000000001);
#34548=CIRCLE('',#107801,0.127);
#34549=CIRCLE('',#107802,0.126999999999999);
#34550=CIRCLE('',#107803,0.127);
#34551=CIRCLE('',#107805,0.127000000000001);
#34552=CIRCLE('',#107808,0.127000000000001);
#34553=CIRCLE('',#107810,0.127000000000002);
#34554=CIRCLE('',#107812,0.127);
#34555=CIRCLE('',#107813,0.127);
#34556=CIRCLE('',#107814,0.127);
#34557=CIRCLE('',#107816,0.127);
#34558=CIRCLE('',#107819,0.126999999999998);
#34559=CIRCLE('',#107823,0.127000000000001);
#34560=CIRCLE('',#107824,0.126999999999999);
#34561=CIRCLE('',#107826,0.126999999999999);
#34562=CIRCLE('',#107828,0.127000000000004);
#34563=CIRCLE('',#107829,0.127);
#34564=CIRCLE('',#107830,0.126999999999998);
#34565=CIRCLE('',#107832,0.126999999999999);
#34566=CIRCLE('',#107835,0.126999999999999);
#34567=CIRCLE('',#107837,0.127);
#34568=CIRCLE('',#107839,0.127);
#34569=CIRCLE('',#107840,0.126999999999997);
#34570=CIRCLE('',#107841,0.126999999999997);
#34571=CIRCLE('',#107843,0.127000000000001);
#34572=CIRCLE('',#107845,0.126999999999997);
#34573=CIRCLE('',#107846,0.127000000000003);
#34574=CIRCLE('',#107847,0.126999999999999);
#34575=CIRCLE('',#107849,0.127);
#34576=CIRCLE('',#107852,0.127000000000002);
#34577=CIRCLE('',#107854,0.127000000000002);
#34578=CIRCLE('',#107856,0.127000000000003);
#34579=CIRCLE('',#107857,0.126999999999999);
#34580=CIRCLE('',#107858,0.127000000000004);
#34581=CIRCLE('',#107860,0.126999999999999);
#34582=CIRCLE('',#107863,0.126999999999998);
#34583=CIRCLE('',#107867,0.127);
#34584=CIRCLE('',#107868,0.127);
#34585=CIRCLE('',#107870,0.127);
#34586=CIRCLE('',#107872,0.127);
#34587=CIRCLE('',#107873,0.127000000000003);
#34588=CIRCLE('',#107874,0.127000000000002);
#34589=CIRCLE('',#107876,0.126999999999998);
#34590=CIRCLE('',#107879,0.127000000000003);
#34591=CIRCLE('',#107881,0.127);
#34592=CIRCLE('',#107883,0.126999999999999);
#34593=CIRCLE('',#107884,0.127000000000001);
#34594=CIRCLE('',#107885,0.126999999999998);
#34595=CIRCLE('',#107887,0.127000000000002);
#34596=CIRCLE('',#107889,0.126999999999997);
#34597=CIRCLE('',#107890,0.127000000000004);
#34598=CIRCLE('',#107891,0.127);
#34599=CIRCLE('',#107893,0.127000000000001);
#34600=CIRCLE('',#107896,0.126999999999998);
#34601=CIRCLE('',#107898,0.127000000000002);
#34602=CIRCLE('',#107900,0.127);
#34603=CIRCLE('',#107901,0.127);
#34604=CIRCLE('',#107902,0.127);
#34605=CIRCLE('',#107904,0.127);
#34606=CIRCLE('',#107907,0.127000000000002);
#34607=CIRCLE('',#107911,0.127000000000002);
#34608=CIRCLE('',#107912,0.127);
#34609=CIRCLE('',#107914,0.127);
#34610=CIRCLE('',#107916,0.127);
#34611=CIRCLE('',#107917,0.126999999999998);
#34612=CIRCLE('',#107918,0.127000000000002);
#34613=CIRCLE('',#107920,0.126999999999999);
#34614=CIRCLE('',#107923,0.126999999999999);
#34615=CIRCLE('',#107925,0.127);
#34616=CIRCLE('',#107927,0.127000000000003);
#34617=CIRCLE('',#107928,0.127000000000002);
#34618=CIRCLE('',#107929,0.126999999999998);
#34619=CIRCLE('',#107931,0.126999999999999);
#34620=CIRCLE('',#107933,0.126999999999997);
#34621=CIRCLE('',#107934,0.127000000000001);
#34622=CIRCLE('',#107935,0.127);
#34623=CIRCLE('',#107937,0.127);
#34624=CIRCLE('',#107940,0.127000000000002);
#34625=CIRCLE('',#107942,0.127000000000001);
#34626=CIRCLE('',#107944,0.126999999999998);
#34627=CIRCLE('',#107945,0.127);
#34628=CIRCLE('',#107946,0.127);
#34629=CIRCLE('',#107948,0.127);
#34630=CIRCLE('',#107951,0.127000000000002);
#34631=CIRCLE('',#107955,0.127000000000001);
#34632=CIRCLE('',#107956,0.127);
#34633=CIRCLE('',#107958,0.126999999999999);
#34634=CIRCLE('',#107960,0.127000000000004);
#34635=CIRCLE('',#107961,0.127000000000001);
#34636=CIRCLE('',#107962,0.126999999999999);
#34637=CIRCLE('',#107964,0.126999999999999);
#34638=CIRCLE('',#107967,0.126999999999995);
#34639=CIRCLE('',#107969,0.127);
#34640=CIRCLE('',#107971,0.126999999999998);
#34641=CIRCLE('',#107972,0.127000000000002);
#34642=CIRCLE('',#107973,0.126999999999998);
#34643=CIRCLE('',#107975,0.126999999999999);
#34644=CIRCLE('',#107977,0.127000000000003);
#34645=CIRCLE('',#107978,0.127000000000001);
#34646=CIRCLE('',#107979,0.126999999999999);
#34647=CIRCLE('',#107981,0.127000000000003);
#34648=CIRCLE('',#107984,0.127);
#34649=CIRCLE('',#107986,0.127000000000001);
#34650=CIRCLE('',#107988,0.127000000000003);
#34651=CIRCLE('',#107989,0.126999999999999);
#34652=CIRCLE('',#107990,0.126999999999999);
#34653=CIRCLE('',#107992,0.126999999999999);
#34654=CIRCLE('',#107995,0.126999999999997);
#34655=CIRCLE('',#107999,0.127);
#34656=CIRCLE('',#108000,0.127);
#34657=CIRCLE('',#108002,0.127);
#34658=CIRCLE('',#108004,0.127);
#34659=CIRCLE('',#108005,0.127);
#34660=CIRCLE('',#108006,0.126999999999999);
#34661=CIRCLE('',#108008,0.126999999999999);
#34662=CIRCLE('',#108011,0.127000000000002);
#34663=CIRCLE('',#108013,0.127);
#34664=CIRCLE('',#108015,0.126999999999999);
#34665=CIRCLE('',#108016,0.126999999999997);
#34666=CIRCLE('',#108017,0.126999999999999);
#34667=CIRCLE('',#108019,0.126999999999999);
#34668=CIRCLE('',#108021,0.126999999999998);
#34669=CIRCLE('',#108022,0.127);
#34670=CIRCLE('',#108023,0.127);
#34671=CIRCLE('',#108025,0.126999999999999);
#34672=CIRCLE('',#108028,0.126999999999999);
#34673=CIRCLE('',#108030,0.127);
#34674=CIRCLE('',#108032,0.127000000000003);
#34675=CIRCLE('',#108033,0.127);
#34676=CIRCLE('',#108034,0.127);
#34677=CIRCLE('',#108036,0.127);
#34678=CIRCLE('',#108039,0.127);
#34679=CIRCLE('',#108043,0.126999999999998);
#34680=CIRCLE('',#108044,0.127000000000001);
#34681=CIRCLE('',#108046,0.127000000000001);
#34682=CIRCLE('',#108048,0.127000000000001);
#34683=CIRCLE('',#108049,0.127000000000002);
#34684=CIRCLE('',#108050,0.127000000000003);
#34685=CIRCLE('',#108052,0.126999999999998);
#34686=CIRCLE('',#108055,0.127000000000001);
#34687=CIRCLE('',#108057,0.127000000000001);
#34688=CIRCLE('',#108059,0.127000000000001);
#34689=CIRCLE('',#108060,0.126999999999999);
#34690=CIRCLE('',#108061,0.126999999999999);
#34691=CIRCLE('',#108063,0.126999999999999);
#34692=CIRCLE('',#108065,0.127000000000002);
#34693=CIRCLE('',#108066,0.126999999999997);
#34694=CIRCLE('',#108067,0.127000000000001);
#34695=CIRCLE('',#108069,0.127000000000001);
#34696=CIRCLE('',#108072,0.126999999999998);
#34697=CIRCLE('',#108074,0.126999999999999);
#34698=CIRCLE('',#108076,0.126999999999998);
#34699=CIRCLE('',#108077,0.127000000000001);
#34700=CIRCLE('',#108078,0.127000000000001);
#34701=CIRCLE('',#108080,0.127000000000001);
#34702=CIRCLE('',#108083,0.127000000000003);
#34703=CIRCLE('',#108087,0.127000000000003);
#34704=CIRCLE('',#108088,0.127000000000002);
#34705=CIRCLE('',#108090,0.126999999999999);
#34706=CIRCLE('',#108092,0.126999999999999);
#34707=CIRCLE('',#108093,0.127000000000002);
#34708=CIRCLE('',#108094,0.127000000000001);
#34709=CIRCLE('',#108096,0.126999999999998);
#34710=CIRCLE('',#108099,0.127);
#34711=CIRCLE('',#108101,0.127);
#34712=CIRCLE('',#108103,0.126999999999998);
#34713=CIRCLE('',#108104,0.127);
#34714=CIRCLE('',#108105,0.126999999999998);
#34715=CIRCLE('',#108107,0.126999999999997);
#34716=CIRCLE('',#108109,0.127);
#34717=CIRCLE('',#108110,0.127);
#34718=CIRCLE('',#108111,0.126999999999999);
#34719=CIRCLE('',#108113,0.127000000000003);
#34720=CIRCLE('',#108116,0.127000000000003);
#34721=CIRCLE('',#108118,0.126999999999999);
#34722=CIRCLE('',#108120,0.127);
#34723=CIRCLE('',#108121,0.126999999999999);
#34724=CIRCLE('',#108122,0.126999999999999);
#34725=CIRCLE('',#108124,0.126999999999999);
#34726=CIRCLE('',#108127,0.127000000000002);
#34727=CIRCLE('',#108131,0.127);
#34728=CIRCLE('',#108132,0.126999999999999);
#34729=CIRCLE('',#108134,0.126999999999999);
#34730=CIRCLE('',#108136,0.126999999999999);
#34731=CIRCLE('',#108137,0.126999999999997);
#34732=CIRCLE('',#108138,0.127000000000003);
#34733=CIRCLE('',#108140,0.127000000000002);
#34734=CIRCLE('',#108143,0.126999999999997);
#34735=CIRCLE('',#108145,0.126999999999999);
#34736=CIRCLE('',#108147,0.127000000000003);
#34737=CIRCLE('',#108148,0.127000000000002);
#34738=CIRCLE('',#108149,0.127000000000001);
#34739=CIRCLE('',#108151,0.127000000000003);
#34740=CIRCLE('',#108153,0.127000000000002);
#34741=CIRCLE('',#108154,0.127);
#34742=CIRCLE('',#108155,0.126999999999999);
#34743=CIRCLE('',#108157,0.127000000000002);
#34744=CIRCLE('',#108160,0.127000000000002);
#34745=CIRCLE('',#108162,0.126999999999997);
#34746=CIRCLE('',#108164,0.126999999999997);
#34747=CIRCLE('',#108165,0.126999999999999);
#34748=CIRCLE('',#108166,0.126999999999999);
#34749=CIRCLE('',#108168,0.126999999999999);
#34750=CIRCLE('',#108171,0.127);
#34751=CIRCLE('',#108175,0.127000000000003);
#34752=CIRCLE('',#108176,0.127);
#34753=CIRCLE('',#108178,0.127);
#34754=CIRCLE('',#108180,0.127);
#34755=CIRCLE('',#108181,0.127000000000001);
#34756=CIRCLE('',#108182,0.127);
#34757=CIRCLE('',#108184,0.126999999999999);
#34758=CIRCLE('',#108187,0.127000000000002);
#34759=CIRCLE('',#108189,0.127);
#34760=CIRCLE('',#108191,0.127000000000004);
#34761=CIRCLE('',#108192,0.127000000000002);
#34762=CIRCLE('',#108193,0.126999999999999);
#34763=CIRCLE('',#108195,0.126999999999999);
#34764=CIRCLE('',#108197,0.126999999999998);
#34765=CIRCLE('',#108198,0.126999999999997);
#34766=CIRCLE('',#108199,0.127);
#34767=CIRCLE('',#108201,0.127);
#34768=CIRCLE('',#108204,0.127);
#34769=CIRCLE('',#108206,0.127000000000001);
#34770=CIRCLE('',#108208,0.126999999999998);
#34771=CIRCLE('',#108209,0.127);
#34772=CIRCLE('',#108210,0.127);
#34773=CIRCLE('',#108212,0.127);
#34774=CIRCLE('',#108215,0.126999999999999);
#34775=CIRCLE('',#108219,0.126999999999999);
#34776=CIRCLE('',#108220,0.127);
#34777=CIRCLE('',#108222,0.127);
#34778=CIRCLE('',#108224,0.127);
#34779=CIRCLE('',#108225,0.126999999999999);
#34780=CIRCLE('',#108226,0.127);
#34781=CIRCLE('',#108228,0.127000000000005);
#34782=CIRCLE('',#108231,0.127000000000002);
#34783=CIRCLE('',#108233,0.127);
#34784=CIRCLE('',#108235,0.127000000000002);
#34785=CIRCLE('',#108236,0.127);
#34786=CIRCLE('',#108237,0.126999999999998);
#34787=CIRCLE('',#108239,0.126999999999998);
#34788=CIRCLE('',#108241,0.126999999999999);
#34789=CIRCLE('',#108242,0.127000000000002);
#34790=CIRCLE('',#108243,0.127);
#34791=CIRCLE('',#108245,0.127000000000002);
#34792=CIRCLE('',#108248,0.126999999999998);
#34793=CIRCLE('',#108250,0.127000000000003);
#34794=CIRCLE('',#108252,0.127);
#34795=CIRCLE('',#108253,0.127);
#34796=CIRCLE('',#108254,0.127);
#34797=CIRCLE('',#108256,0.127);
#34798=CIRCLE('',#108259,0.127);
#34799=CIRCLE('',#108263,0.127000000000003);
#34800=CIRCLE('',#108264,0.127);
#34801=CIRCLE('',#108266,0.127);
#34802=CIRCLE('',#108268,0.127);
#34803=CIRCLE('',#108269,0.127);
#34804=CIRCLE('',#108270,0.126999999999999);
#34805=CIRCLE('',#108272,0.126999999999998);
#34806=CIRCLE('',#108275,0.127000000000004);
#34807=CIRCLE('',#108277,0.127);
#34808=CIRCLE('',#108279,0.127000000000002);
#34809=CIRCLE('',#108280,0.126999999999998);
#34810=CIRCLE('',#108281,0.126999999999999);
#34811=CIRCLE('',#108283,0.127);
#34812=CIRCLE('',#108285,0.127000000000002);
#34813=CIRCLE('',#108286,0.127);
#34814=CIRCLE('',#108287,0.127);
#34815=CIRCLE('',#108289,0.126999999999997);
#34816=CIRCLE('',#108292,0.126999999999999);
#34817=CIRCLE('',#108294,0.127000000000002);
#34818=CIRCLE('',#108296,0.127000000000002);
#34819=CIRCLE('',#108297,0.127);
#34820=CIRCLE('',#108298,0.127);
#34821=CIRCLE('',#108300,0.127);
#34822=CIRCLE('',#108303,0.127000000000002);
#34823=CIRCLE('',#108307,0.127);
#34824=CIRCLE('',#108308,0.126999999999999);
#34825=CIRCLE('',#108310,0.126999999999999);
#34826=CIRCLE('',#108312,0.126999999999999);
#34827=CIRCLE('',#108313,0.127000000000001);
#34828=CIRCLE('',#108314,0.127);
#34829=CIRCLE('',#108316,0.127000000000002);
#34830=CIRCLE('',#108319,0.126999999999997);
#34831=CIRCLE('',#108321,0.126999999999999);
#34832=CIRCLE('',#108323,0.126999999999997);
#34833=CIRCLE('',#108324,0.127);
#34834=CIRCLE('',#108325,0.127000000000003);
#34835=CIRCLE('',#108327,0.127000000000002);
#34836=CIRCLE('',#108329,0.127);
#34837=CIRCLE('',#108330,0.127000000000002);
#34838=CIRCLE('',#108331,0.126999999999999);
#34839=CIRCLE('',#108333,0.127000000000001);
#34840=CIRCLE('',#108336,0.127000000000002);
#34841=CIRCLE('',#108338,0.126999999999998);
#34842=CIRCLE('',#108340,0.127000000000002);
#34843=CIRCLE('',#108341,0.126999999999999);
#34844=CIRCLE('',#108342,0.126999999999999);
#34845=CIRCLE('',#108344,0.126999999999999);
#34846=CIRCLE('',#108347,0.127000000000002);
#34847=CIRCLE('',#108351,0.127000000000002);
#34848=CIRCLE('',#108352,0.126999999999999);
#34849=CIRCLE('',#108354,0.126999999999999);
#34850=CIRCLE('',#108356,0.127);
#34851=CIRCLE('',#108357,0.127);
#34852=CIRCLE('',#108358,0.127000000000001);
#34853=CIRCLE('',#108360,0.126999999999998);
#34854=CIRCLE('',#108363,0.126999999999998);
#34855=CIRCLE('',#108365,0.126999999999999);
#34856=CIRCLE('',#108367,0.127);
#34857=CIRCLE('',#108368,0.127);
#34858=CIRCLE('',#108369,0.127000000000002);
#34859=CIRCLE('',#108371,0.127000000000003);
#34860=CIRCLE('',#108373,0.127000000000002);
#34861=CIRCLE('',#108374,0.126999999999997);
#34862=CIRCLE('',#108375,0.126999999999999);
#34863=CIRCLE('',#108377,0.127);
#34864=CIRCLE('',#108380,0.126999999999997);
#34865=CIRCLE('',#108382,0.127000000000002);
#34866=CIRCLE('',#108384,0.126999999999999);
#34867=CIRCLE('',#108385,0.126999999999999);
#34868=CIRCLE('',#108386,0.126999999999999);
#34869=CIRCLE('',#108388,0.126999999999999);
#34870=CIRCLE('',#108391,0.127000000000001);
#34871=CIRCLE('',#108395,0.126999999999998);
#34872=CIRCLE('',#108396,0.127000000000001);
#34873=CIRCLE('',#108398,0.127000000000001);
#34874=CIRCLE('',#108400,0.127000000000001);
#34875=CIRCLE('',#108401,0.127000000000001);
#34876=CIRCLE('',#108402,0.127);
#34877=CIRCLE('',#108404,0.126999999999999);
#34878=CIRCLE('',#108407,0.127000000000002);
#34879=CIRCLE('',#108409,0.127000000000001);
#34880=CIRCLE('',#108411,0.127000000000001);
#34881=CIRCLE('',#108412,0.126999999999998);
#34882=CIRCLE('',#108413,0.126999999999998);
#34883=CIRCLE('',#108415,0.126999999999999);
#34884=CIRCLE('',#108417,0.127);
#34885=CIRCLE('',#108418,0.127000000000002);
#34886=CIRCLE('',#108419,0.127000000000001);
#34887=CIRCLE('',#108421,0.126999999999998);
#34888=CIRCLE('',#108424,0.126999999999999);
#34889=CIRCLE('',#108426,0.126999999999998);
#34890=CIRCLE('',#108428,0.127000000000002);
#34891=CIRCLE('',#108429,0.127000000000001);
#34892=CIRCLE('',#108430,0.127000000000001);
#34893=CIRCLE('',#108432,0.127000000000001);
#34894=CIRCLE('',#108435,0.126999999999998);
#34895=CIRCLE('',#108439,0.127);
#34896=CIRCLE('',#108440,0.127);
#34897=CIRCLE('',#108442,0.127000000000003);
#34898=CIRCLE('',#108444,0.127);
#34899=CIRCLE('',#108445,0.127000000000001);
#34900=CIRCLE('',#108446,0.127);
#34901=CIRCLE('',#108448,0.127);
#34902=CIRCLE('',#108451,0.126999999999998);
#34903=CIRCLE('',#108453,0.127);
#34904=CIRCLE('',#108455,0.127000000000002);
#34905=CIRCLE('',#108456,0.127000000000001);
#34906=CIRCLE('',#108457,0.127);
#34907=CIRCLE('',#108459,0.127);
#34908=CIRCLE('',#108461,0.127000000000002);
#34909=CIRCLE('',#108462,0.126999999999999);
#34910=CIRCLE('',#108463,0.127);
#34911=CIRCLE('',#108465,0.127);
#34912=CIRCLE('',#108468,0.127);
#34913=CIRCLE('',#108470,0.127000000000001);
#34914=CIRCLE('',#108472,0.127);
#34915=CIRCLE('',#108473,0.127);
#34916=CIRCLE('',#108474,0.127);
#34917=CIRCLE('',#108476,0.127);
#34918=CIRCLE('',#108479,0.127);
#34919=CIRCLE('',#108483,0.127000000000001);
#34920=CIRCLE('',#108484,0.127000000000004);
#34921=CIRCLE('',#108486,0.126999999999999);
#34922=CIRCLE('',#108488,0.127000000000004);
#34923=CIRCLE('',#108489,0.127);
#34924=CIRCLE('',#108490,0.126999999999999);
#34925=CIRCLE('',#108492,0.126999999999999);
#34926=CIRCLE('',#108495,0.126999999999998);
#34927=CIRCLE('',#108497,0.127000000000004);
#34928=CIRCLE('',#108499,0.126999999999995);
#34929=CIRCLE('',#108500,0.127000000000003);
#34930=CIRCLE('',#108501,0.127000000000001);
#34931=CIRCLE('',#108503,0.127);
#34932=CIRCLE('',#108505,0.126999999999999);
#34933=CIRCLE('',#108506,0.127000000000003);
#34934=CIRCLE('',#108507,0.126999999999999);
#34935=CIRCLE('',#108509,0.127);
#34936=CIRCLE('',#108512,0.127000000000001);
#34937=CIRCLE('',#108514,0.126999999999998);
#34938=CIRCLE('',#108516,0.127000000000002);
#34939=CIRCLE('',#108517,0.126999999999999);
#34940=CIRCLE('',#108518,0.126999999999999);
#34941=CIRCLE('',#108520,0.126999999999999);
#34942=CIRCLE('',#108523,0.126999999999999);
#34943=CIRCLE('',#108527,0.127);
#34944=CIRCLE('',#108528,0.127);
#34945=CIRCLE('',#108530,0.127);
#34946=CIRCLE('',#108532,0.127);
#34947=CIRCLE('',#108533,0.126999999999998);
#34948=CIRCLE('',#108534,0.127000000000002);
#34949=CIRCLE('',#108536,0.126999999999999);
#34950=CIRCLE('',#108539,0.126999999999998);
#34951=CIRCLE('',#108541,0.127);
#34952=CIRCLE('',#108543,0.126999999999998);
#34953=CIRCLE('',#108544,0.127);
#34954=CIRCLE('',#108545,0.126999999999999);
#34955=CIRCLE('',#108547,0.127);
#34956=CIRCLE('',#108549,0.126999999999997);
#34957=CIRCLE('',#108550,0.127);
#34958=CIRCLE('',#108551,0.127);
#34959=CIRCLE('',#108553,0.126999999999996);
#34960=CIRCLE('',#108556,0.127000000000003);
#34961=CIRCLE('',#108558,0.126999999999998);
#34962=CIRCLE('',#108560,0.127000000000002);
#34963=CIRCLE('',#108561,0.127);
#34964=CIRCLE('',#108562,0.127);
#34965=CIRCLE('',#108564,0.127);
#34966=CIRCLE('',#108567,0.127000000000002);
#34967=CIRCLE('',#108571,0.127);
#34968=CIRCLE('',#108572,0.127);
#34969=CIRCLE('',#108574,0.127);
#34970=CIRCLE('',#108576,0.127);
#34971=CIRCLE('',#108577,0.127000000000003);
#34972=CIRCLE('',#108578,0.127000000000003);
#34973=CIRCLE('',#108580,0.127000000000003);
#34974=CIRCLE('',#108583,0.126999999999999);
#34975=CIRCLE('',#108585,0.127);
#34976=CIRCLE('',#108587,0.127000000000003);
#34977=CIRCLE('',#108588,0.127000000000003);
#34978=CIRCLE('',#108589,0.127000000000002);
#34979=CIRCLE('',#108591,0.126999999999998);
#34980=CIRCLE('',#108593,0.126999999999998);
#34981=CIRCLE('',#108594,0.127000000000001);
#34982=CIRCLE('',#108595,0.127);
#34983=CIRCLE('',#108597,0.127);
#34984=CIRCLE('',#108600,0.127000000000002);
#34985=CIRCLE('',#108602,0.126999999999999);
#34986=CIRCLE('',#108604,0.127000000000002);
#34987=CIRCLE('',#108605,0.127);
#34988=CIRCLE('',#108606,0.127);
#34989=CIRCLE('',#108608,0.127);
#34990=CIRCLE('',#108611,0.127000000000002);
#34991=CIRCLE('',#108615,0.127000000000002);
#34992=CIRCLE('',#108616,0.127000000000004);
#34993=CIRCLE('',#108618,0.127000000000004);
#34994=CIRCLE('',#108620,0.127);
#34995=CIRCLE('',#108621,0.127);
#34996=CIRCLE('',#108622,0.126999999999998);
#34997=CIRCLE('',#108624,0.127);
#34998=CIRCLE('',#108627,0.126999999999995);
#34999=CIRCLE('',#108629,0.127000000000004);
#35000=CIRCLE('',#108631,0.126999999999998);
#35001=CIRCLE('',#108632,0.126999999999999);
#35002=CIRCLE('',#108633,0.127);
#35003=CIRCLE('',#108635,0.126999999999999);
#35004=CIRCLE('',#108637,0.127000000000001);
#35005=CIRCLE('',#108638,0.127);
#35006=CIRCLE('',#108639,0.127000000000004);
#35007=CIRCLE('',#108641,0.127000000000003);
#35008=CIRCLE('',#108644,0.127000000000001);
#35009=CIRCLE('',#108646,0.127);
#35010=CIRCLE('',#108648,0.127000000000002);
#35011=CIRCLE('',#108649,0.127000000000004);
#35012=CIRCLE('',#108650,0.127);
#35013=CIRCLE('',#108652,0.127000000000004);
#35014=CIRCLE('',#108655,0.126999999999999);
#35015=CIRCLE('',#108659,0.127);
#35016=CIRCLE('',#108660,0.127);
#35017=CIRCLE('',#108662,0.127);
#35018=CIRCLE('',#108664,0.127);
#35019=CIRCLE('',#108665,0.126999999999999);
#35020=CIRCLE('',#108666,0.127);
#35021=CIRCLE('',#108668,0.126999999999999);
#35022=CIRCLE('',#108671,0.127000000000002);
#35023=CIRCLE('',#108673,0.126999999999999);
#35024=CIRCLE('',#108675,0.127000000000002);
#35025=CIRCLE('',#108676,0.127000000000001);
#35026=CIRCLE('',#108677,0.127);
#35027=CIRCLE('',#108679,0.126999999999998);
#35028=CIRCLE('',#108681,0.126999999999999);
#35029=CIRCLE('',#108682,0.127);
#35030=CIRCLE('',#108683,0.127);
#35031=CIRCLE('',#108685,0.126999999999998);
#35032=CIRCLE('',#108688,0.127000000000002);
#35033=CIRCLE('',#108690,0.126999999999997);
#35034=CIRCLE('',#108692,0.127000000000001);
#35035=CIRCLE('',#108693,0.127);
#35036=CIRCLE('',#108694,0.127);
#35037=CIRCLE('',#108696,0.127);
#35038=CIRCLE('',#108699,0.126999999999998);
#35039=CIRCLE('',#108703,0.127);
#35040=CIRCLE('',#108704,0.127000000000001);
#35041=CIRCLE('',#108706,0.127000000000001);
#35042=CIRCLE('',#108708,0.127000000000001);
#35043=CIRCLE('',#108709,0.127);
#35044=CIRCLE('',#108710,0.127000000000002);
#35045=CIRCLE('',#108712,0.126999999999999);
#35046=CIRCLE('',#108715,0.127000000000002);
#35047=CIRCLE('',#108717,0.127000000000001);
#35048=CIRCLE('',#108719,0.127000000000001);
#35049=CIRCLE('',#108720,0.127000000000001);
#35050=CIRCLE('',#108721,0.127);
#35051=CIRCLE('',#108723,0.126999999999998);
#35052=CIRCLE('',#108725,0.126999999999999);
#35053=CIRCLE('',#108726,0.127000000000003);
#35054=CIRCLE('',#108727,0.127000000000001);
#35055=CIRCLE('',#108729,0.127000000000001);
#35056=CIRCLE('',#108732,0.126999999999999);
#35057=CIRCLE('',#108734,0.126999999999998);
#35058=CIRCLE('',#108736,0.126999999999999);
#35059=CIRCLE('',#108737,0.127000000000001);
#35060=CIRCLE('',#108738,0.127000000000001);
#35061=CIRCLE('',#108740,0.127000000000001);
#35062=CIRCLE('',#108743,0.127000000000001);
#35063=CIRCLE('',#108747,0.126999999999998);
#35064=CIRCLE('',#108748,0.126999999999999);
#35065=CIRCLE('',#108750,0.126999999999999);
#35066=CIRCLE('',#108752,0.126999999999999);
#35067=CIRCLE('',#108753,0.127);
#35068=CIRCLE('',#108754,0.127000000000001);
#35069=CIRCLE('',#108756,0.126999999999997);
#35070=CIRCLE('',#108759,0.127);
#35071=CIRCLE('',#108761,0.127);
#35072=CIRCLE('',#108763,0.126999999999998);
#35073=CIRCLE('',#108764,0.127);
#35074=CIRCLE('',#108765,0.126999999999998);
#35075=CIRCLE('',#108767,0.126999999999998);
#35076=CIRCLE('',#108769,0.127000000000002);
#35077=CIRCLE('',#108770,0.126999999999999);
#35078=CIRCLE('',#108771,0.126999999999999);
#35079=CIRCLE('',#108773,0.127000000000002);
#35080=CIRCLE('',#108776,0.126999999999997);
#35081=CIRCLE('',#108778,0.127);
#35082=CIRCLE('',#108780,0.127);
#35083=CIRCLE('',#108781,0.126999999999999);
#35084=CIRCLE('',#108782,0.127);
#35085=CIRCLE('',#108784,0.126999999999999);
#35086=CIRCLE('',#108787,0.127000000000002);
#35087=CIRCLE('',#108791,0.127);
#35088=CIRCLE('',#108792,0.127000000000001);
#35089=CIRCLE('',#108794,0.126999999999999);
#35090=CIRCLE('',#108796,0.127000000000001);
#35091=CIRCLE('',#108797,0.127000000000003);
#35092=CIRCLE('',#108798,0.127);
#35093=CIRCLE('',#108800,0.127000000000001);
#35094=CIRCLE('',#108803,0.126999999999997);
#35095=CIRCLE('',#108805,0.126999999999999);
#35096=CIRCLE('',#108807,0.126999999999997);
#35097=CIRCLE('',#108808,0.126999999999999);
#35098=CIRCLE('',#108809,0.127);
#35099=CIRCLE('',#108811,0.127000000000002);
#35100=CIRCLE('',#108813,0.126999999999999);
#35101=CIRCLE('',#108814,0.127);
#35102=CIRCLE('',#108815,0.126999999999999);
#35103=CIRCLE('',#108817,0.127000000000002);
#35104=CIRCLE('',#108820,0.127000000000003);
#35105=CIRCLE('',#108822,0.127);
#35106=CIRCLE('',#108824,0.126999999999997);
#35107=CIRCLE('',#108825,0.126999999999999);
#35108=CIRCLE('',#108826,0.126999999999999);
#35109=CIRCLE('',#108828,0.126999999999999);
#35110=CIRCLE('',#108831,0.127);
#35111=CIRCLE('',#108835,0.127000000000003);
#35112=CIRCLE('',#108836,0.127);
#35113=CIRCLE('',#108838,0.127);
#35114=CIRCLE('',#108840,0.127);
#35115=CIRCLE('',#108841,0.126999999999997);
#35116=CIRCLE('',#108842,0.127);
#35117=CIRCLE('',#108844,0.126999999999999);
#35118=CIRCLE('',#108847,0.127000000000002);
#35119=CIRCLE('',#108849,0.127);
#35120=CIRCLE('',#108851,0.127000000000004);
#35121=CIRCLE('',#108852,0.127000000000003);
#35122=CIRCLE('',#108853,0.126999999999998);
#35123=CIRCLE('',#108855,0.126999999999999);
#35124=CIRCLE('',#108857,0.126999999999998);
#35125=CIRCLE('',#108858,0.126999999999997);
#35126=CIRCLE('',#108859,0.127);
#35127=CIRCLE('',#108861,0.127);
#35128=CIRCLE('',#108864,0.127);
#35129=CIRCLE('',#108866,0.127000000000002);
#35130=CIRCLE('',#108868,0.126999999999998);
#35131=CIRCLE('',#108869,0.127);
#35132=CIRCLE('',#108870,0.127);
#35133=CIRCLE('',#108872,0.127);
#35134=CIRCLE('',#108875,0.127000000000001);
#35135=CIRCLE('',#108879,0.127);
#35136=CIRCLE('',#108880,0.127);
#35137=CIRCLE('',#108882,0.127);
#35138=CIRCLE('',#108884,0.127);
#35139=CIRCLE('',#108885,0.126999999999999);
#35140=CIRCLE('',#108886,0.127);
#35141=CIRCLE('',#108888,0.127000000000005);
#35142=CIRCLE('',#108892,0.127);
#35143=CIRCLE('',#108893,0.127);
#35144=CIRCLE('',#108894,0.127000000000005);
#35145=CIRCLE('',#108896,0.126999999999998);
#35146=CIRCLE('',#108898,0.126999999999999);
#35147=CIRCLE('',#108899,0.127);
#35148=CIRCLE('',#108902,0.126999999999998);
#35149=CIRCLE('',#108904,0.127);
#35150=CIRCLE('',#108906,0.127);
#35151=CIRCLE('',#108907,0.127);
#35152=CIRCLE('',#108908,0.127);
#35153=CIRCLE('',#108910,0.127);
#35154=CIRCLE('',#108913,0.127000000000001);
#35155=CIRCLE('',#108917,0.126999999999997);
#35156=CIRCLE('',#108918,0.127);
#35157=CIRCLE('',#108920,0.127);
#35158=CIRCLE('',#108922,0.127);
#35159=CIRCLE('',#108923,0.126999999999998);
#35160=CIRCLE('',#108924,0.126999999999999);
#35161=CIRCLE('',#108926,0.126999999999998);
#35162=CIRCLE('',#108929,0.127000000000004);
#35163=CIRCLE('',#108931,0.127);
#35164=CIRCLE('',#108933,0.127000000000002);
#35165=CIRCLE('',#108934,0.126999999999998);
#35166=CIRCLE('',#108935,0.126999999999998);
#35167=CIRCLE('',#108937,0.127);
#35168=CIRCLE('',#108939,0.126999999999998);
#35169=CIRCLE('',#108940,0.127);
#35170=CIRCLE('',#108941,0.127);
#35171=CIRCLE('',#108943,0.126999999999997);
#35172=CIRCLE('',#108946,0.126999999999999);
#35173=CIRCLE('',#108948,0.127000000000002);
#35174=CIRCLE('',#108950,0.127000000000003);
#35175=CIRCLE('',#108951,0.127);
#35176=CIRCLE('',#108952,0.127);
#35177=CIRCLE('',#108954,0.127);
#35178=CIRCLE('',#108957,0.127000000000001);
#35179=CIRCLE('',#108961,0.127);
#35180=CIRCLE('',#108962,0.126999999999999);
#35181=CIRCLE('',#108964,0.126999999999999);
#35182=CIRCLE('',#108966,0.126999999999999);
#35183=CIRCLE('',#108967,0.127000000000003);
#35184=CIRCLE('',#108968,0.127);
#35185=CIRCLE('',#108970,0.127000000000001);
#35186=CIRCLE('',#108973,0.126999999999997);
#35187=CIRCLE('',#108975,0.126999999999999);
#35188=CIRCLE('',#108977,0.126999999999997);
#35189=CIRCLE('',#108978,0.126999999999998);
#35190=CIRCLE('',#108979,0.127000000000002);
#35191=CIRCLE('',#108981,0.127000000000003);
#35192=CIRCLE('',#108983,0.127000000000001);
#35193=CIRCLE('',#108984,0.127000000000002);
#35194=CIRCLE('',#108985,0.126999999999999);
#35195=CIRCLE('',#108987,0.127000000000001);
#35196=CIRCLE('',#108990,0.127000000000003);
#35197=CIRCLE('',#108992,0.127000000000002);
#35198=CIRCLE('',#108994,0.127000000000003);
#35199=CIRCLE('',#108995,0.126999999999999);
#35200=CIRCLE('',#108996,0.126999999999999);
#35201=CIRCLE('',#108998,0.126999999999999);
#35202=CIRCLE('',#109001,0.127000000000001);
#35203=CIRCLE('',#109005,0.127000000000002);
#35204=CIRCLE('',#109006,0.126999999999999);
#35205=CIRCLE('',#109008,0.126999999999999);
#35206=CIRCLE('',#109010,0.127000000000002);
#35207=CIRCLE('',#109011,0.126999999999999);
#35208=CIRCLE('',#109012,0.127);
#35209=CIRCLE('',#109014,0.126999999999997);
#35210=CIRCLE('',#109017,0.126999999999999);
#35211=CIRCLE('',#109019,0.127000000000002);
#35212=CIRCLE('',#109021,0.127000000000001);
#35213=CIRCLE('',#109022,0.127);
#35214=CIRCLE('',#109023,0.127);
#35215=CIRCLE('',#109025,0.126999999999998);
#35216=CIRCLE('',#109027,0.126999999999999);
#35217=CIRCLE('',#109028,0.126999999999997);
#35218=CIRCLE('',#109029,0.126999999999999);
#35219=CIRCLE('',#109031,0.127);
#35220=CIRCLE('',#109034,0.127000000000003);
#35221=CIRCLE('',#109036,0.127);
#35222=CIRCLE('',#109038,0.126999999999999);
#35223=CIRCLE('',#109039,0.126999999999999);
#35224=CIRCLE('',#109040,0.126999999999999);
#35225=CIRCLE('',#109042,0.126999999999999);
#35226=CIRCLE('',#109045,0.127000000000002);
#35227=CIRCLE('',#109049,0.126999999999998);
#35228=CIRCLE('',#109050,0.127000000000001);
#35229=CIRCLE('',#109052,0.127000000000001);
#35230=CIRCLE('',#109054,0.127000000000001);
#35231=CIRCLE('',#109055,0.126999999999999);
#35232=CIRCLE('',#109056,0.127000000000003);
#35233=CIRCLE('',#109058,0.127);
#35234=CIRCLE('',#109061,0.127000000000002);
#35235=CIRCLE('',#109063,0.127000000000001);
#35236=CIRCLE('',#109065,0.127000000000001);
#35237=CIRCLE('',#109066,0.127000000000001);
#35238=CIRCLE('',#109067,0.127000000000001);
#35239=CIRCLE('',#109069,0.127);
#35240=CIRCLE('',#109071,0.127);
#35241=CIRCLE('',#109072,0.127000000000002);
#35242=CIRCLE('',#109073,0.127000000000001);
#35243=CIRCLE('',#109075,0.126999999999998);
#35244=CIRCLE('',#109078,0.126999999999998);
#35245=CIRCLE('',#109080,0.127000000000001);
#35246=CIRCLE('',#109082,0.127000000000003);
#35247=CIRCLE('',#109083,0.127000000000001);
#35248=CIRCLE('',#109084,0.127000000000001);
#35249=CIRCLE('',#109086,0.127000000000001);
#35250=CIRCLE('',#109089,0.127000000000002);
#35251=CIRCLE('',#109093,0.127000000000001);
#35252=CIRCLE('',#109094,0.127);
#35253=CIRCLE('',#109096,0.127000000000003);
#35254=CIRCLE('',#109098,0.127);
#35255=CIRCLE('',#109099,0.126999999999998);
#35256=CIRCLE('',#109100,0.126999999999999);
#35257=CIRCLE('',#109102,0.127000000000001);
#35258=CIRCLE('',#109105,0.127000000000002);
#35259=CIRCLE('',#109107,0.127);
#35260=CIRCLE('',#109109,0.127000000000002);
#35261=CIRCLE('',#109110,0.126999999999999);
#35262=CIRCLE('',#109111,0.127000000000001);
#35263=CIRCLE('',#109113,0.127000000000001);
#35264=CIRCLE('',#109115,0.126999999999999);
#35265=CIRCLE('',#109116,0.126999999999999);
#35266=CIRCLE('',#109117,0.127);
#35267=CIRCLE('',#109119,0.127000000000001);
#35268=CIRCLE('',#109122,0.127);
#35269=CIRCLE('',#109124,0.127);
#35270=CIRCLE('',#109126,0.127);
#35271=CIRCLE('',#109127,0.127);
#35272=CIRCLE('',#109128,0.127);
#35273=CIRCLE('',#109130,0.127);
#35274=CIRCLE('',#109133,0.126999999999998);
#35275=CIRCLE('',#109137,0.127000000000001);
#35276=CIRCLE('',#109138,0.127000000000004);
#35277=CIRCLE('',#109140,0.126999999999999);
#35278=CIRCLE('',#109142,0.127000000000004);
#35279=CIRCLE('',#109143,0.126999999999999);
#35280=CIRCLE('',#109144,0.126999999999999);
#35281=CIRCLE('',#109146,0.126999999999999);
#35282=CIRCLE('',#109149,0.126999999999998);
#35283=CIRCLE('',#109151,0.127000000000003);
#35284=CIRCLE('',#109153,0.126999999999995);
#35285=CIRCLE('',#109154,0.127);
#35286=CIRCLE('',#109155,0.126999999999999);
#35287=CIRCLE('',#109157,0.127);
#35288=CIRCLE('',#109159,0.127000000000001);
#35289=CIRCLE('',#109160,0.127000000000003);
#35290=CIRCLE('',#109161,0.126999999999999);
#35291=CIRCLE('',#109163,0.127);
#35292=CIRCLE('',#109166,0.126999999999999);
#35293=CIRCLE('',#109168,0.127000000000001);
#35294=CIRCLE('',#109170,0.126999999999997);
#35295=CIRCLE('',#109171,0.126999999999999);
#35296=CIRCLE('',#109172,0.126999999999999);
#35297=CIRCLE('',#109174,0.126999999999999);
#35298=CIRCLE('',#109177,0.126999999999997);
#35299=CIRCLE('',#109181,0.126999999999999);
#35300=CIRCLE('',#109182,0.127);
#35301=CIRCLE('',#109184,0.127);
#35302=CIRCLE('',#109186,0.127);
#35303=CIRCLE('',#109187,0.126999999999997);
#35304=CIRCLE('',#109188,0.127000000000002);
#35305=CIRCLE('',#109190,0.127000000000003);
#35306=CIRCLE('',#109193,0.127000000000003);
#35307=CIRCLE('',#109195,0.127);
#35308=CIRCLE('',#109197,0.126999999999998);
#35309=CIRCLE('',#109198,0.127);
#35310=CIRCLE('',#109199,0.126999999999997);
#35311=CIRCLE('',#109201,0.127000000000002);
#35312=CIRCLE('',#109203,0.127000000000002);
#35313=CIRCLE('',#109204,0.127);
#35314=CIRCLE('',#109205,0.127);
#35315=CIRCLE('',#109207,0.126999999999996);
#35316=CIRCLE('',#109210,0.126999999999999);
#35317=CIRCLE('',#109212,0.126999999999997);
#35318=CIRCLE('',#109214,0.127000000000002);
#35319=CIRCLE('',#109215,0.127);
#35320=CIRCLE('',#109216,0.127);
#35321=CIRCLE('',#109218,0.127);
#35322=CIRCLE('',#109221,0.127000000000002);
#35323=CIRCLE('',#109225,0.127);
#35324=CIRCLE('',#109226,0.127);
#35325=CIRCLE('',#109228,0.127);
#35326=CIRCLE('',#109230,0.127);
#35327=CIRCLE('',#109231,0.127000000000002);
#35328=CIRCLE('',#109232,0.127000000000003);
#35329=CIRCLE('',#109234,0.126999999999998);
#35330=CIRCLE('',#109237,0.126999999999999);
#35331=CIRCLE('',#109239,0.127);
#35332=CIRCLE('',#109241,0.127000000000003);
#35333=CIRCLE('',#109242,0.126999999999998);
#35334=CIRCLE('',#109243,0.126999999999998);
#35335=CIRCLE('',#109245,0.126999999999999);
#35336=CIRCLE('',#109247,0.126999999999998);
#35337=CIRCLE('',#109248,0.127000000000001);
#35338=CIRCLE('',#109249,0.127);
#35339=CIRCLE('',#109251,0.127);
#35340=CIRCLE('',#109254,0.127000000000002);
#35341=CIRCLE('',#109256,0.126999999999997);
#35342=CIRCLE('',#109258,0.126999999999998);
#35343=CIRCLE('',#109259,0.127);
#35344=CIRCLE('',#109260,0.127);
#35345=CIRCLE('',#109262,0.127);
#35346=CIRCLE('',#109265,0.127000000000003);
#35347=CIRCLE('',#109269,0.127000000000002);
#35348=CIRCLE('',#109270,0.127000000000004);
#35349=CIRCLE('',#109272,0.127000000000004);
#35350=CIRCLE('',#109274,0.127000000000004);
#35351=CIRCLE('',#109275,0.127);
#35352=CIRCLE('',#109276,0.127000000000001);
#35353=CIRCLE('',#109278,0.126999999999999);
#35354=CIRCLE('',#109281,0.126999999999995);
#35355=CIRCLE('',#109283,0.127000000000004);
#35356=CIRCLE('',#109285,0.126999999999998);
#35357=CIRCLE('',#109286,0.127000000000002);
#35358=CIRCLE('',#109287,0.126999999999997);
#35359=CIRCLE('',#109289,0.127);
#35360=CIRCLE('',#109291,0.127);
#35361=CIRCLE('',#109292,0.127);
#35362=CIRCLE('',#109293,0.127000000000004);
#35363=CIRCLE('',#109295,0.127000000000003);
#35364=CIRCLE('',#109298,0.127000000000002);
#35365=CIRCLE('',#109300,0.126999999999999);
#35366=CIRCLE('',#109302,0.126999999999999);
#35367=CIRCLE('',#109303,0.127000000000004);
#35368=CIRCLE('',#109304,0.126999999999999);
#35369=CIRCLE('',#109306,0.127000000000004);
#35370=CIRCLE('',#109309,0.126999999999997);
#35371=CIRCLE('',#109313,0.127000000000002);
#35372=CIRCLE('',#109314,0.127);
#35373=CIRCLE('',#109316,0.127);
#35374=CIRCLE('',#109318,0.127);
#35375=CIRCLE('',#109319,0.126999999999998);
#35376=CIRCLE('',#109320,0.127000000000001);
#35377=CIRCLE('',#109322,0.126999999999999);
#35378=CIRCLE('',#109325,0.127000000000002);
#35379=CIRCLE('',#109327,0.127);
#35380=CIRCLE('',#109329,0.127000000000002);
#35381=CIRCLE('',#109330,0.127000000000002);
#35382=CIRCLE('',#109331,0.126999999999999);
#35383=CIRCLE('',#109333,0.127);
#35384=CIRCLE('',#109335,0.127000000000001);
#35385=CIRCLE('',#109336,0.127);
#35386=CIRCLE('',#109337,0.127000000000003);
#35387=CIRCLE('',#109339,0.126999999999999);
#35388=CIRCLE('',#109342,0.127000000000002);
#35389=CIRCLE('',#109344,0.126999999999998);
#35390=CIRCLE('',#109346,0.127000000000001);
#35391=CIRCLE('',#109347,0.127);
#35392=CIRCLE('',#109348,0.127);
#35393=CIRCLE('',#109350,0.127);
#35394=CIRCLE('',#109353,0.127000000000002);
#35395=CIRCLE('',#109357,0.126999999999999);
#35396=CIRCLE('',#109358,0.127000000000001);
#35397=CIRCLE('',#109360,0.127000000000001);
#35398=CIRCLE('',#109362,0.127000000000001);
#35399=CIRCLE('',#109363,0.127000000000002);
#35400=CIRCLE('',#109364,0.127000000000002);
#35401=CIRCLE('',#109366,0.126999999999999);
#35402=CIRCLE('',#109369,0.126999999999999);
#35403=CIRCLE('',#109371,0.127000000000001);
#35404=CIRCLE('',#109373,0.127000000000002);
#35405=CIRCLE('',#109374,0.127000000000001);
#35406=CIRCLE('',#109375,0.126999999999999);
#35407=CIRCLE('',#109377,0.126999999999999);
#35408=CIRCLE('',#109379,0.127);
#35409=CIRCLE('',#109380,0.127000000000003);
#35410=CIRCLE('',#109381,0.127000000000001);
#35411=CIRCLE('',#109383,0.127000000000001);
#35412=CIRCLE('',#109386,0.126999999999999);
#35413=CIRCLE('',#109388,0.127000000000002);
#35414=CIRCLE('',#109390,0.127);
#35415=CIRCLE('',#109391,0.127000000000001);
#35416=CIRCLE('',#109392,0.127000000000001);
#35417=CIRCLE('',#109394,0.127000000000001);
#35418=CIRCLE('',#109397,0.127000000000002);
#35419=CIRCLE('',#109401,0.126999999999998);
#35420=CIRCLE('',#109402,0.127);
#35421=CIRCLE('',#109404,0.127);
#35422=CIRCLE('',#109406,0.126999999999999);
#35423=CIRCLE('',#109407,0.127);
#35424=CIRCLE('',#109408,0.127000000000001);
#35425=CIRCLE('',#109410,0.126999999999998);
#35426=CIRCLE('',#109413,0.127);
#35427=CIRCLE('',#109415,0.127);
#35428=CIRCLE('',#109417,0.126999999999998);
#35429=CIRCLE('',#109418,0.126999999999997);
#35430=CIRCLE('',#109419,0.127000000000003);
#35431=CIRCLE('',#109421,0.126999999999999);
#35432=CIRCLE('',#109423,0.127000000000002);
#35433=CIRCLE('',#109424,0.126999999999999);
#35434=CIRCLE('',#109425,0.127);
#35435=CIRCLE('',#109427,0.127000000000002);
#35436=CIRCLE('',#109430,0.126999999999999);
#35437=CIRCLE('',#109432,0.127000000000003);
#35438=CIRCLE('',#109434,0.127);
#35439=CIRCLE('',#109435,0.127);
#35440=CIRCLE('',#109436,0.127);
#35441=CIRCLE('',#109438,0.127);
#35442=CIRCLE('',#109441,0.127);
#35443=CIRCLE('',#109445,0.127);
#35444=CIRCLE('',#109446,0.126999999999999);
#35445=CIRCLE('',#109448,0.126999999999999);
#35446=CIRCLE('',#109450,0.126999999999999);
#35447=CIRCLE('',#109451,0.127000000000001);
#35448=CIRCLE('',#109452,0.126999999999999);
#35449=CIRCLE('',#109454,0.126999999999997);
#35450=CIRCLE('',#109457,0.127000000000003);
#35451=CIRCLE('',#109459,0.126999999999999);
#35452=CIRCLE('',#109461,0.126999999999996);
#35453=CIRCLE('',#109462,0.127);
#35454=CIRCLE('',#109463,0.127000000000001);
#35455=CIRCLE('',#109465,0.126999999999997);
#35456=CIRCLE('',#109467,0.127000000000002);
#35457=CIRCLE('',#109468,0.127);
#35458=CIRCLE('',#109469,0.126999999999999);
#35459=CIRCLE('',#109471,0.127000000000002);
#35460=CIRCLE('',#109474,0.126999999999998);
#35461=CIRCLE('',#109476,0.127);
#35462=CIRCLE('',#109478,0.126999999999999);
#35463=CIRCLE('',#109479,0.126999999999999);
#35464=CIRCLE('',#109480,0.126999999999999);
#35465=CIRCLE('',#109482,0.126999999999999);
#35466=CIRCLE('',#109485,0.127);
#35467=CIRCLE('',#109489,0.126999999999998);
#35468=CIRCLE('',#109490,0.127);
#35469=CIRCLE('',#109492,0.127);
#35470=CIRCLE('',#109494,0.127);
#35471=CIRCLE('',#109495,0.127000000000003);
#35472=CIRCLE('',#109496,0.126999999999999);
#35473=CIRCLE('',#109498,0.127);
#35474=CIRCLE('',#109501,0.127000000000002);
#35475=CIRCLE('',#109503,0.127);
#35476=CIRCLE('',#109505,0.127000000000004);
#35477=CIRCLE('',#109506,0.127);
#35478=CIRCLE('',#109507,0.126999999999999);
#35479=CIRCLE('',#109509,0.127);
#35480=CIRCLE('',#109511,0.127000000000001);
#35481=CIRCLE('',#109512,0.126999999999997);
#35482=CIRCLE('',#109513,0.127);
#35483=CIRCLE('',#109515,0.127);
#35484=CIRCLE('',#109518,0.127000000000001);
#35485=CIRCLE('',#109520,0.127000000000003);
#35486=CIRCLE('',#109522,0.126999999999999);
#35487=CIRCLE('',#109523,0.127);
#35488=CIRCLE('',#109524,0.127);
#35489=CIRCLE('',#109526,0.127);
#35490=CIRCLE('',#109529,0.126999999999998);
#35491=CIRCLE('',#109533,0.127);
#35492=CIRCLE('',#109534,0.127);
#35493=CIRCLE('',#109536,0.127);
#35494=CIRCLE('',#109538,0.127);
#35495=CIRCLE('',#109539,0.126999999999999);
#35496=CIRCLE('',#109540,0.126999999999999);
#35497=CIRCLE('',#109542,0.127000000000004);
#35498=CIRCLE('',#109546,0.127);
#35499=CIRCLE('',#109547,0.127);
#35500=CIRCLE('',#109548,0.127000000000004);
#35501=CIRCLE('',#109550,0.126999999999999);
#35502=CIRCLE('',#109552,0.126999999999999);
#35503=CIRCLE('',#109553,0.127);
#35504=CIRCLE('',#109556,0.126999999999999);
#35505=CIRCLE('',#109558,0.126999999999999);
#35506=CIRCLE('',#109560,0.127);
#35507=CIRCLE('',#109561,0.127);
#35508=CIRCLE('',#109562,0.127);
#35509=CIRCLE('',#109564,0.127);
#35510=CIRCLE('',#109567,0.126999999999999);
#35511=CIRCLE('',#109571,0.126999999999998);
#35512=CIRCLE('',#109572,0.127);
#35513=CIRCLE('',#109574,0.127);
#35514=CIRCLE('',#109576,0.127);
#35515=CIRCLE('',#109577,0.126999999999997);
#35516=CIRCLE('',#109578,0.127);
#35517=CIRCLE('',#109580,0.126999999999998);
#35518=CIRCLE('',#109583,0.127000000000004);
#35519=CIRCLE('',#109585,0.127);
#35520=CIRCLE('',#109587,0.127000000000002);
#35521=CIRCLE('',#109588,0.126999999999998);
#35522=CIRCLE('',#109589,0.126999999999998);
#35523=CIRCLE('',#109591,0.127);
#35524=CIRCLE('',#109593,0.127000000000002);
#35525=CIRCLE('',#109594,0.127);
#35526=CIRCLE('',#109595,0.127);
#35527=CIRCLE('',#109597,0.126999999999997);
#35528=CIRCLE('',#109600,0.127);
#35529=CIRCLE('',#109602,0.127000000000002);
#35530=CIRCLE('',#109604,0.126999999999997);
#35531=CIRCLE('',#109605,0.127);
#35532=CIRCLE('',#109606,0.127);
#35533=CIRCLE('',#109608,0.127);
#35534=CIRCLE('',#109611,0.126999999999998);
#35535=CIRCLE('',#109615,0.127);
#35536=CIRCLE('',#109616,0.126999999999999);
#35537=CIRCLE('',#109618,0.126999999999999);
#35538=CIRCLE('',#109620,0.126999999999999);
#35539=CIRCLE('',#109621,0.127000000000002);
#35540=CIRCLE('',#109622,0.126999999999999);
#35541=CIRCLE('',#109624,0.127);
#35542=CIRCLE('',#109627,0.126999999999997);
#35543=CIRCLE('',#109629,0.127000000000001);
#35544=CIRCLE('',#109631,0.126999999999997);
#35545=CIRCLE('',#109632,0.126999999999998);
#35546=CIRCLE('',#109633,0.126999999999999);
#35547=CIRCLE('',#109635,0.127000000000003);
#35548=CIRCLE('',#109637,0.127000000000002);
#35549=CIRCLE('',#109638,0.127000000000002);
#35550=CIRCLE('',#109639,0.126999999999999);
#35551=CIRCLE('',#109641,0.127000000000001);
#35552=CIRCLE('',#109644,0.127000000000002);
#35553=CIRCLE('',#109646,0.127);
#35554=CIRCLE('',#109648,0.126999999999998);
#35555=CIRCLE('',#109649,0.126999999999999);
#35556=CIRCLE('',#109650,0.126999999999999);
#35557=CIRCLE('',#109652,0.126999999999999);
#35558=CIRCLE('',#109655,0.126999999999999);
#35559=CIRCLE('',#109659,0.126999999999997);
#35560=CIRCLE('',#109660,0.126999999999999);
#35561=CIRCLE('',#109662,0.126999999999999);
#35562=CIRCLE('',#109664,0.127);
#35563=CIRCLE('',#109665,0.126999999999998);
#35564=CIRCLE('',#109666,0.126999999999997);
#35565=CIRCLE('',#109668,0.127000000000002);
#35566=CIRCLE('',#109671,0.126999999999998);
#35567=CIRCLE('',#109673,0.126999999999999);
#35568=CIRCLE('',#109675,0.127000000000001);
#35569=CIRCLE('',#109676,0.127000000000002);
#35570=CIRCLE('',#109677,0.127000000000001);
#35571=CIRCLE('',#109679,0.126999999999997);
#35572=CIRCLE('',#109681,0.126999999999999);
#35573=CIRCLE('',#109682,0.126999999999997);
#35574=CIRCLE('',#109683,0.126999999999999);
#35575=CIRCLE('',#109685,0.127);
#35576=CIRCLE('',#109688,0.126999999999999);
#35577=CIRCLE('',#109690,0.126999999999999);
#35578=CIRCLE('',#109692,0.127);
#35579=CIRCLE('',#109693,0.126999999999999);
#35580=CIRCLE('',#109694,0.126999999999999);
#35581=CIRCLE('',#109696,0.126999999999999);
#35582=CIRCLE('',#109699,0.127000000000001);
#35583=CIRCLE('',#109703,0.126999999999999);
#35584=CIRCLE('',#109704,0.127000000000001);
#35585=CIRCLE('',#109706,0.127000000000001);
#35586=CIRCLE('',#109708,0.127000000000001);
#35587=CIRCLE('',#109709,0.127000000000001);
#35588=CIRCLE('',#109710,0.127000000000003);
#35589=CIRCLE('',#109712,0.127000000000003);
#35590=CIRCLE('',#109715,0.127000000000002);
#35591=CIRCLE('',#109717,0.127000000000001);
#35592=CIRCLE('',#109719,0.127000000000001);
#35593=CIRCLE('',#109720,0.126999999999998);
#35594=CIRCLE('',#109721,0.126999999999998);
#35595=CIRCLE('',#109723,0.126999999999999);
#35596=CIRCLE('',#109725,0.127000000000002);
#35597=CIRCLE('',#109726,0.127000000000001);
#35598=CIRCLE('',#109727,0.127000000000001);
#35599=CIRCLE('',#109729,0.126999999999998);
#35600=CIRCLE('',#109732,0.127);
#35601=CIRCLE('',#109734,0.127000000000003);
#35602=CIRCLE('',#109736,0.126999999999997);
#35603=CIRCLE('',#109737,0.127000000000001);
#35604=CIRCLE('',#109738,0.127000000000001);
#35605=CIRCLE('',#109740,0.127000000000001);
#35606=CIRCLE('',#109743,0.127000000000002);
#35607=CIRCLE('',#109747,0.127000000000001);
#35608=CIRCLE('',#109748,0.127);
#35609=CIRCLE('',#109750,0.127000000000003);
#35610=CIRCLE('',#109752,0.127);
#35611=CIRCLE('',#109753,0.127);
#35612=CIRCLE('',#109754,0.126999999999999);
#35613=CIRCLE('',#109756,0.126999999999999);
#35614=CIRCLE('',#109759,0.126999999999998);
#35615=CIRCLE('',#109761,0.127);
#35616=CIRCLE('',#109763,0.126999999999996);
#35617=CIRCLE('',#109764,0.127000000000001);
#35618=CIRCLE('',#109765,0.126999999999998);
#35619=CIRCLE('',#109767,0.127000000000001);
#35620=CIRCLE('',#109769,0.127000000000002);
#35621=CIRCLE('',#109770,0.126999999999999);
#35622=CIRCLE('',#109771,0.127);
#35623=CIRCLE('',#109773,0.127000000000001);
#35624=CIRCLE('',#109776,0.126999999999999);
#35625=CIRCLE('',#109778,0.127000000000002);
#35626=CIRCLE('',#109780,0.127000000000001);
#35627=CIRCLE('',#109781,0.127);
#35628=CIRCLE('',#109782,0.127);
#35629=CIRCLE('',#109784,0.127);
#35630=CIRCLE('',#109787,0.126999999999997);
#35631=CIRCLE('',#109791,0.127000000000002);
#35632=CIRCLE('',#109792,0.126999999999999);
#35633=CIRCLE('',#109794,0.126999999999999);
#35634=CIRCLE('',#109796,0.127000000000004);
#35635=CIRCLE('',#109797,0.126999999999999);
#35636=CIRCLE('',#109798,0.126999999999998);
#35637=CIRCLE('',#109800,0.126999999999999);
#35638=CIRCLE('',#109803,0.126999999999998);
#35639=CIRCLE('',#109805,0.127000000000004);
#35640=CIRCLE('',#109807,0.127);
#35641=CIRCLE('',#109808,0.126999999999998);
#35642=CIRCLE('',#109809,0.126999999999998);
#35643=CIRCLE('',#109811,0.127000000000002);
#35644=CIRCLE('',#109813,0.126999999999997);
#35645=CIRCLE('',#109814,0.127000000000003);
#35646=CIRCLE('',#109815,0.126999999999999);
#35647=CIRCLE('',#109817,0.127);
#35648=CIRCLE('',#109820,0.127000000000001);
#35649=CIRCLE('',#109822,0.126999999999997);
#35650=CIRCLE('',#109824,0.127000000000001);
#35651=CIRCLE('',#109825,0.126999999999999);
#35652=CIRCLE('',#109826,0.126999999999999);
#35653=CIRCLE('',#109828,0.126999999999999);
#35654=CIRCLE('',#109831,0.126999999999998);
#35655=CIRCLE('',#109835,0.126999999999999);
#35656=CIRCLE('',#109836,0.127);
#35657=CIRCLE('',#109838,0.127);
#35658=CIRCLE('',#109840,0.127);
#35659=CIRCLE('',#109841,0.127000000000002);
#35660=CIRCLE('',#109842,0.127000000000001);
#35661=CIRCLE('',#109844,0.126999999999998);
#35662=CIRCLE('',#109847,0.126999999999998);
#35663=CIRCLE('',#109849,0.127);
#35664=CIRCLE('',#109851,0.126999999999998);
#35665=CIRCLE('',#109852,0.127);
#35666=CIRCLE('',#109853,0.126999999999999);
#35667=CIRCLE('',#109855,0.127000000000002);
#35668=CIRCLE('',#109857,0.127000000000001);
#35669=CIRCLE('',#109858,0.127);
#35670=CIRCLE('',#109859,0.127);
#35671=CIRCLE('',#109861,0.126999999999996);
#35672=CIRCLE('',#109864,0.126999999999998);
#35673=CIRCLE('',#109866,0.127000000000001);
#35674=CIRCLE('',#109868,0.127000000000001);
#35675=CIRCLE('',#109869,0.127);
#35676=CIRCLE('',#109870,0.127);
#35677=CIRCLE('',#109872,0.127);
#35678=CIRCLE('',#109875,0.127000000000001);
#35679=CIRCLE('',#109879,0.127);
#35680=CIRCLE('',#109880,0.127);
#35681=CIRCLE('',#109882,0.127);
#35682=CIRCLE('',#109884,0.127);
#35683=CIRCLE('',#109885,0.127000000000002);
#35684=CIRCLE('',#109886,0.127000000000002);
#35685=CIRCLE('',#109888,0.126999999999998);
#35686=CIRCLE('',#109891,0.126999999999999);
#35687=CIRCLE('',#109893,0.127);
#35688=CIRCLE('',#109895,0.127000000000003);
#35689=CIRCLE('',#109896,0.126999999999997);
#35690=CIRCLE('',#109897,0.126999999999998);
#35691=CIRCLE('',#109899,0.126999999999999);
#35692=CIRCLE('',#109901,0.127);
#35693=CIRCLE('',#109902,0.127000000000001);
#35694=CIRCLE('',#109903,0.127);
#35695=CIRCLE('',#109905,0.127);
#35696=CIRCLE('',#109908,0.127000000000002);
#35697=CIRCLE('',#109910,0.126999999999997);
#35698=CIRCLE('',#109912,0.126999999999997);
#35699=CIRCLE('',#109913,0.127);
#35700=CIRCLE('',#109914,0.127);
#35701=CIRCLE('',#109916,0.127);
#35702=CIRCLE('',#109919,0.127000000000002);
#35703=CIRCLE('',#109923,0.127000000000002);
#35704=CIRCLE('',#109924,0.127000000000004);
#35705=CIRCLE('',#109926,0.127000000000004);
#35706=CIRCLE('',#109928,0.127000000000004);
#35707=CIRCLE('',#109929,0.127);
#35708=CIRCLE('',#109930,0.126999999999998);
#35709=CIRCLE('',#109932,0.127);
#35710=CIRCLE('',#109935,0.127000000000001);
#35711=CIRCLE('',#109937,0.127000000000004);
#35712=CIRCLE('',#109939,0.126999999999998);
#35713=CIRCLE('',#109940,0.126999999999999);
#35714=CIRCLE('',#109941,0.127);
#35715=CIRCLE('',#109943,0.126999999999999);
#35716=CIRCLE('',#109945,0.127000000000002);
#35717=CIRCLE('',#109946,0.126999999999996);
#35718=CIRCLE('',#109947,0.127000000000004);
#35719=CIRCLE('',#109949,0.127000000000003);
#35720=CIRCLE('',#109952,0.127);
#35721=CIRCLE('',#109954,0.127000000000002);
#35722=CIRCLE('',#109956,0.127);
#35723=CIRCLE('',#109957,0.127000000000004);
#35724=CIRCLE('',#109958,0.127);
#35725=CIRCLE('',#109960,0.127000000000004);
#35726=CIRCLE('',#109963,0.126999999999997);
#35727=CIRCLE('',#109967,0.127);
#35728=CIRCLE('',#109968,0.127);
#35729=CIRCLE('',#109970,0.127);
#35730=CIRCLE('',#109972,0.126999999999999);
#35731=CIRCLE('',#109973,0.126999999999999);
#35732=CIRCLE('',#109974,0.126999999999999);
#35733=CIRCLE('',#109976,0.126999999999998);
#35734=CIRCLE('',#109979,0.127000000000002);
#35735=CIRCLE('',#109981,0.127);
#35736=CIRCLE('',#109983,0.127000000000002);
#35737=CIRCLE('',#109984,0.127000000000002);
#35738=CIRCLE('',#109985,0.127);
#35739=CIRCLE('',#109987,0.126999999999999);
#35740=CIRCLE('',#109989,0.127);
#35741=CIRCLE('',#109990,0.127);
#35742=CIRCLE('',#109991,0.127);
#35743=CIRCLE('',#109993,0.126999999999998);
#35744=CIRCLE('',#109996,0.127);
#35745=CIRCLE('',#109998,0.127000000000002);
#35746=CIRCLE('',#110000,0.127000000000002);
#35747=CIRCLE('',#110001,0.127);
#35748=CIRCLE('',#110002,0.127);
#35749=CIRCLE('',#110004,0.127);
#35750=CIRCLE('',#110007,0.127000000000003);
#35751=CIRCLE('',#110011,0.126999999999998);
#35752=CIRCLE('',#110012,0.127000000000001);
#35753=CIRCLE('',#110014,0.127000000000001);
#35754=CIRCLE('',#110016,0.127000000000001);
#35755=CIRCLE('',#110017,0.127);
#35756=CIRCLE('',#110018,0.127000000000002);
#35757=CIRCLE('',#110020,0.126999999999999);
#35758=CIRCLE('',#110023,0.127000000000001);
#35759=CIRCLE('',#110025,0.126999999999998);
#35760=CIRCLE('',#110027,0.127000000000001);
#35761=CIRCLE('',#110028,0.127);
#35762=CIRCLE('',#110029,0.126999999999999);
#35763=CIRCLE('',#110031,0.126999999999998);
#35764=CIRCLE('',#110033,0.126999999999999);
#35765=CIRCLE('',#110034,0.127000000000003);
#35766=CIRCLE('',#110035,0.127000000000001);
#35767=CIRCLE('',#110037,0.127000000000001);
#35768=CIRCLE('',#110040,0.127);
#35769=CIRCLE('',#110042,0.126999999999999);
#35770=CIRCLE('',#110044,0.126999999999999);
#35771=CIRCLE('',#110045,0.127000000000001);
#35772=CIRCLE('',#110046,0.127000000000001);
#35773=CIRCLE('',#110048,0.127000000000001);
#35774=CIRCLE('',#110051,0.127000000000002);
#35775=CIRCLE('',#110055,0.127000000000001);
#35776=CIRCLE('',#110056,0.127);
#35777=CIRCLE('',#110058,0.127);
#35778=CIRCLE('',#110060,0.127);
#35779=CIRCLE('',#110061,0.127000000000001);
#35780=CIRCLE('',#110062,0.126999999999997);
#35781=CIRCLE('',#110064,0.126999999999999);
#35782=CIRCLE('',#110067,0.127);
#35783=CIRCLE('',#110069,0.127);
#35784=CIRCLE('',#110071,0.126999999999998);
#35785=CIRCLE('',#110072,0.127);
#35786=CIRCLE('',#110073,0.126999999999998);
#35787=CIRCLE('',#110075,0.126999999999998);
#35788=CIRCLE('',#110077,0.127);
#35789=CIRCLE('',#110078,0.126999999999999);
#35790=CIRCLE('',#110079,0.127);
#35791=CIRCLE('',#110081,0.127000000000002);
#35792=CIRCLE('',#110084,0.126999999999998);
#35793=CIRCLE('',#110086,0.127);
#35794=CIRCLE('',#110088,0.126999999999999);
#35795=CIRCLE('',#110089,0.127);
#35796=CIRCLE('',#110090,0.127);
#35797=CIRCLE('',#110092,0.127);
#35798=CIRCLE('',#110095,0.127000000000002);
#35799=CIRCLE('',#110099,0.127);
#35800=CIRCLE('',#110100,0.126999999999999);
#35801=CIRCLE('',#110102,0.126999999999999);
#35802=CIRCLE('',#110104,0.126999999999999);
#35803=CIRCLE('',#110105,0.127000000000002);
#35804=CIRCLE('',#110106,0.127000000000002);
#35805=CIRCLE('',#110108,0.127000000000001);
#35806=CIRCLE('',#110111,0.127000000000003);
#35807=CIRCLE('',#110113,0.126999999999999);
#35808=CIRCLE('',#110115,0.126999999999996);
#35809=CIRCLE('',#110116,0.127000000000003);
#35810=CIRCLE('',#110117,0.127);
#35811=CIRCLE('',#110119,0.127000000000003);
#35812=CIRCLE('',#110121,0.127000000000002);
#35813=CIRCLE('',#110122,0.127);
#35814=CIRCLE('',#110123,0.126999999999999);
#35815=CIRCLE('',#110125,0.127000000000002);
#35816=CIRCLE('',#110128,0.127000000000003);
#35817=CIRCLE('',#110130,0.126999999999998);
#35818=CIRCLE('',#110132,0.126999999999998);
#35819=CIRCLE('',#110133,0.126999999999999);
#35820=CIRCLE('',#110134,0.126999999999999);
#35821=CIRCLE('',#110136,0.126999999999999);
#35822=CIRCLE('',#110139,0.127);
#35823=CIRCLE('',#110143,0.126999999999997);
#35824=CIRCLE('',#110144,0.127);
#35825=CIRCLE('',#110146,0.127);
#35826=CIRCLE('',#110148,0.127);
#35827=CIRCLE('',#110149,0.126999999999997);
#35828=CIRCLE('',#110150,0.127);
#35829=CIRCLE('',#110152,0.126999999999999);
#35830=CIRCLE('',#110155,0.127000000000002);
#35831=CIRCLE('',#110157,0.127);
#35832=CIRCLE('',#110159,0.127000000000004);
#35833=CIRCLE('',#110160,0.127);
#35834=CIRCLE('',#110161,0.126999999999999);
#35835=CIRCLE('',#110163,0.127);
#35836=CIRCLE('',#110165,0.126999999999998);
#35837=CIRCLE('',#110166,0.126999999999997);
#35838=CIRCLE('',#110167,0.127);
#35839=CIRCLE('',#110169,0.127);
#35840=CIRCLE('',#110172,0.127);
#35841=CIRCLE('',#110174,0.127);
#35842=CIRCLE('',#110176,0.126999999999998);
#35843=CIRCLE('',#110177,0.127);
#35844=CIRCLE('',#110178,0.127);
#35845=CIRCLE('',#110180,0.127);
#35846=CIRCLE('',#110183,0.126999999999999);
#35847=CIRCLE('',#110186,65.254);
#35848=CIRCLE('',#110187,0.127);
#35849=CIRCLE('',#110188,65.381);
#35850=CIRCLE('',#110190,68.623);
#35851=CIRCLE('',#110191,0.127);
#35852=CIRCLE('',#110192,68.75);
#35853=CIRCLE('',#110194,68.877);
#35854=CIRCLE('',#110195,0.127);
#35855=CIRCLE('',#110196,68.75);
#35856=CIRCLE('',#110197,68.75);
#35857=CIRCLE('',#110199,65.254);
#35858=CIRCLE('',#110202,72.53);
#35859=CIRCLE('',#110203,72.53);
#35860=CIRCLE('',#110208,65.);
#35861=CIRCLE('',#110209,0.0762);
#35862=CIRCLE('',#110210,65.0762);
#35863=CIRCLE('',#110212,65.1778);
#35864=CIRCLE('',#110213,0.0762);
#35865=CIRCLE('',#110214,65.254);
#35866=CIRCLE('',#110216,65.);
#35867=CIRCLE('',#110218,65.254);
#35868=CIRCLE('',#110222,70.625);
#35869=CIRCLE('',#110223,0.8255);
#35870=CIRCLE('',#110224,71.3206076480316);
#35871=CIRCLE('',#110226,77.1551372062631);
#35872=CIRCLE('',#110227,2.53999999999999);
#35873=CIRCLE('',#110228,74.6340699810941);
#35874=CIRCLE('',#110229,2.54);
#35875=CIRCLE('',#110231,25.);
#35876=CIRCLE('',#110232,1.27);
#35877=CIRCLE('',#110233,23.73);
#35878=CIRCLE('',#110234,1.27);
#35879=CIRCLE('',#110236,25.);
#35880=CIRCLE('',#110237,1.27);
#35881=CIRCLE('',#110238,23.73);
#35882=CIRCLE('',#110239,1.27);
#35883=CIRCLE('',#110240,0.634999999999997);
#35884=CIRCLE('',#110241,1.905);
#35885=CIRCLE('',#110242,2.54);
#35886=CIRCLE('',#110243,1.905);
#35887=CIRCLE('',#110244,0.634999999999997);
#35888=CIRCLE('',#110245,1.905);
#35889=CIRCLE('',#110246,2.54);
#35890=CIRCLE('',#110247,1.905);
#35891=CIRCLE('',#110248,0.634999999999997);
#35892=CIRCLE('',#110249,1.905);
#35893=CIRCLE('',#110250,2.54);
#35894=CIRCLE('',#110251,1.905);
#35895=CIRCLE('',#110253,80.);
#35896=CIRCLE('',#110254,81.905);
#35897=CIRCLE('',#110255,1.905);
#35898=CIRCLE('',#110256,0.634999999999997);
#35899=CIRCLE('',#110257,1.905);
#35900=CIRCLE('',#110258,2.54);
#35901=CIRCLE('',#110260,2.54);
#35902=CIRCLE('',#110262,2.54);
#35903=CIRCLE('',#110264,79.9526680629224);
#35904=CIRCLE('',#110265,80.);
#35905=CIRCLE('',#110267,72.53);
#35906=CIRCLE('',#110268,72.53);
#35907=CIRCLE('',#110270,8.4455);
#35908=CIRCLE('',#110271,8.4455);
#35909=CIRCLE('',#110273,8.4455);
#35910=CIRCLE('',#110274,8.4455);
#35911=CIRCLE('',#110276,8.4455);
#35912=CIRCLE('',#110277,8.4455);
#35913=CIRCLE('',#110279,8.4455);
#35914=CIRCLE('',#110280,8.4455);
#35915=CIRCLE('',#110282,80.);
#35916=CIRCLE('',#110284,79.9526680629224);
#35917=CIRCLE('',#110285,79.7261349468031);
#35918=CIRCLE('',#110286,79.7261349468031);
#35919=CIRCLE('',#110287,79.9526680629224);
#35920=CIRCLE('',#110288,79.7261349468031);
#35921=CIRCLE('',#110289,79.9526680629224);
#35922=CIRCLE('',#110290,79.7261349468032);
#35923=CIRCLE('',#110291,79.9526680629224);
#35924=CIRCLE('',#110293,25.);
#35925=CIRCLE('',#110294,25.);
#35926=CIRCLE('',#110295,25.);
#35927=CIRCLE('',#110296,25.);
#35928=CIRCLE('',#110298,25.);
#35929=CIRCLE('',#110299,25.);
#35930=CIRCLE('',#110300,25.);
#35931=CIRCLE('',#110301,25.);
#35932=CIRCLE('',#110306,25.);
#35933=CIRCLE('',#110307,25.);
#35934=CIRCLE('',#110308,25.);
#35935=CIRCLE('',#110310,25.);
#35936=CIRCLE('',#110311,25.);
#35937=CIRCLE('',#110312,25.);
#35938=CIRCLE('',#110315,24.492);
#35939=CIRCLE('',#110316,24.492);
#35940=CIRCLE('',#110319,24.492);
#35941=CIRCLE('',#110320,24.492);
#35942=CIRCLE('',#110323,24.492);
#35943=CIRCLE('',#110324,24.492);
#35944=CIRCLE('',#110327,24.492);
#35945=CIRCLE('',#110328,24.492);
#35946=CIRCLE('',#110331,78.7299999999993);
#35947=CIRCLE('',#110333,7.54337262320408);
#35948=CIRCLE('',#110335,7.54337262320413);
#35949=CIRCLE('',#110337,81.2699999999993);
#35950=CIRCLE('',#110339,80.);
#35951=CIRCLE('',#110340,80.);
#35952=CIRCLE('',#110342,1.27);
#35953=CIRCLE('',#110343,2.54);
#35954=CIRCLE('',#110345,1.27);
#35955=CIRCLE('',#110346,2.54);
#35956=CIRCLE('',#110347,80.);
#35957=CIRCLE('',#110349,80.);
#35958=CIRCLE('',#110351,82.2472021719721);
#35959=CIRCLE('',#110352,23.73);
#35960=CIRCLE('',#110354,80.);
#35961=CIRCLE('',#110356,82.2472021719721);
#35962=CIRCLE('',#110357,23.73);
#35963=CIRCLE('',#110359,80.);
#35964=CIRCLE('',#110360,80.);
#35965=CIRCLE('',#110362,82.2472021719721);
#35966=CIRCLE('',#110364,82.2472021719721);
#35967=CIRCLE('',#110369,26.905);
#35968=CIRCLE('',#110370,26.905);
#35969=CIRCLE('',#110371,81.905);
#35970=CIRCLE('',#110375,26.905);
#35971=CIRCLE('',#110376,26.905);
#35972=CIRCLE('',#110377,0.635);
#35973=CIRCLE('',#110378,81.905);
#35974=CIRCLE('',#110379,0.635);
#35975=CIRCLE('',#110383,26.905);
#35976=CIRCLE('',#110384,26.905);
#35977=CIRCLE('',#110391,6.26916093810295);
#35978=CIRCLE('',#110393,6.26916093808705);
#35979=CIRCLE('',#110397,2.54);
#35980=CIRCLE('',#110398,2.54);
#35981=CIRCLE('',#110400,2.54);
#35982=CIRCLE('',#110401,2.54);
#35983=CIRCLE('',#110403,2.54);
#35984=CIRCLE('',#110405,2.54);
#35985=CIRCLE('',#110407,2.54);
#35986=CIRCLE('',#110409,2.54);
#35987=CIRCLE('',#110410,1.905);
#35988=CIRCLE('',#110411,1.905);
#35989=CIRCLE('',#110413,1.905);
#35990=CIRCLE('',#110415,1.905);
#35991=CIRCLE('',#110417,1.905);
#35992=CIRCLE('',#110418,1.905);
#35993=CIRCLE('',#110420,1.905);
#35994=CIRCLE('',#110423,1.905);
#35995=CIRCLE('',#110425,1.905);
#35996=CIRCLE('',#110427,1.905);
#35997=CIRCLE('',#110429,1.905);
#35998=CIRCLE('',#110432,1.905);
#35999=CIRCLE('',#110434,1.905);
#36000=CIRCLE('',#110437,1.905);
#36001=CIRCLE('',#110439,1.905);
#36002=CIRCLE('',#110442,1.905);
#36003=CIRCLE('',#110444,1.905);
#36004=CIRCLE('',#110445,1.905);
#36005=CIRCLE('',#110446,1.905);
#36006=CIRCLE('',#110448,1.905);
#36007=CIRCLE('',#110450,1.27);
#36008=CIRCLE('',#110452,1.27);
#36009=CIRCLE('',#110459,1.27);
#36010=CIRCLE('',#110461,1.27);
#36011=CIRCLE('',#110463,2.54);
#36012=CIRCLE('',#110465,2.54000000000001);
#36013=CIRCLE('',#110466,2.54);
#36014=CIRCLE('',#110468,2.54);
#36015=CIRCLE('',#110469,2.54);
#36016=CIRCLE('',#110471,2.54);
#36017=CIRCLE('',#110473,2.54);
#36018=CIRCLE('',#110475,2.54);
#36019=CIRCLE('',#110476,1.27);
#36020=CIRCLE('',#110477,1.27);
#36021=CIRCLE('',#110479,1.27);
#36022=CIRCLE('',#110480,1.27);
#36023=CIRCLE('',#110482,1.905);
#36024=CIRCLE('',#110484,1.905);
#36025=CIRCLE('',#110486,1.27);
#36026=CIRCLE('',#110487,1.27);
#36027=CIRCLE('',#110488,1.27);
#36028=CIRCLE('',#110489,1.27);
#36029=CIRCLE('',#110490,1.27);
#36030=CIRCLE('',#110491,1.27);
#36031=CIRCLE('',#110492,1.27);
#36032=CIRCLE('',#110493,1.27);
#36033=CIRCLE('',#110494,1.27);
#36034=CIRCLE('',#110495,1.27);
#36035=CIRCLE('',#110496,1.27);
#36036=CIRCLE('',#110497,1.27);
#36037=CIRCLE('',#110498,1.27);
#36038=CIRCLE('',#110499,1.27);
#36039=CIRCLE('',#110500,1.27);
#36040=CIRCLE('',#110501,1.27);
#36041=CIRCLE('',#110502,1.27);
#36042=CIRCLE('',#110503,2.54);
#36043=CIRCLE('',#110505,2.54);
#36044=CIRCLE('',#110509,0.952500000000001);
#36045=CIRCLE('',#110511,1.905);
#36046=CIRCLE('',#110512,0.0635);
#36047=CIRCLE('',#110513,1.87908163265306);
#36048=CIRCLE('',#110514,1.905);
#36049=CIRCLE('',#110516,1.905);
#36050=CIRCLE('',#110517,0.0635);
#36051=CIRCLE('',#110518,1.8415);
#36052=CIRCLE('',#110519,1.905);
#36053=CIRCLE('',#110520,1.016);
#36054=CIRCLE('',#110521,0.889782955715898);
#36055=CIRCLE('',#110522,1.016);
#36056=CIRCLE('',#110525,1.27);
#36057=CIRCLE('',#110526,1.26090609359413);
#36058=CIRCLE('',#110529,3.17500000000001);
#36059=CIRCLE('',#110532,66.0995441972308);
#36060=CIRCLE('',#110533,0.127);
#36061=CIRCLE('',#110534,66.2265441972308);
#36062=CIRCLE('',#110535,66.0995441972308);
#36063=CIRCLE('',#110537,66.3535441972308);
#36064=CIRCLE('',#110538,0.127);
#36065=CIRCLE('',#110539,66.4805441972308);
#36066=CIRCLE('',#110540,66.4805441972308);
#36067=CIRCLE('',#110543,66.0995441972308);
#36068=CIRCLE('',#110545,66.4805441972308);
#36069=CIRCLE('',#110549,56.0881943187058);
#36070=CIRCLE('',#110550,0.381);
#36071=CIRCLE('',#110551,56.4113006433414);
#36072=CIRCLE('',#110553,50.889);
#36073=CIRCLE('',#110554,0.381);
#36074=CIRCLE('',#110555,51.27);
#36075=CIRCLE('',#110556,51.27);
#36076=CIRCLE('',#110558,50.);
#36077=CIRCLE('',#110559,50.);
#36078=CIRCLE('',#110560,0.381);
#36079=CIRCLE('',#110561,50.381);
#36080=CIRCLE('',#110563,56.5223703788014);
#36081=CIRCLE('',#110564,0.254);
#36082=CIRCLE('',#110565,56.7377745952251);
#36083=CIRCLE('',#110567,57.4087519663171);
#36084=CIRCLE('',#110568,0.254);
#36085=CIRCLE('',#110569,57.6241561827409);
#36086=CIRCLE('',#110571,56.875);
#36087=CIRCLE('',#110572,56.875);
#36088=CIRCLE('',#110576,51.27);
#36089=CIRCLE('',#110578,50.);
#36090=CIRCLE('',#110580,65.);
#36091=CIRCLE('',#110581,65.);
#36092=CIRCLE('',#110595,4.74980000000001);
#36093=CIRCLE('',#110597,4.74980000000001);
#36094=CIRCLE('',#110604,4.74980000000001);
#36095=CIRCLE('',#110606,4.74975596129106);
#36096=CIRCLE('',#110607,4.7227361454377);
#36097=CIRCLE('',#110608,4.84835211827671);
#36098=CIRCLE('',#110609,3.13054999999999);
#36099=CIRCLE('',#110611,4.74980000000001);
#36100=CIRCLE('',#110612,4.72926310421554);
#36101=CIRCLE('',#110613,4.77210660304414);
#36102=CIRCLE('',#110614,4.74980000000001);
#36103=CIRCLE('',#110615,3.98780000000001);
#36104=CIRCLE('',#110619,2.7496306570156);
#36105=CIRCLE('',#110620,2.7496306570156);
#36106=CIRCLE('',#110621,2.7496306570156);
#36107=CIRCLE('',#110622,2.7496306570156);
#36108=CIRCLE('',#110623,2.7496306570156);
#36109=CIRCLE('',#110624,2.7496306570156);
#36110=CIRCLE('',#110640,4.72274603343712);
#36111=CIRCLE('',#110647,4.74980000000001);
#36112=CIRCLE('',#110649,4.74980000000001);
#36113=CIRCLE('',#110656,4.74980000000001);
#36114=CIRCLE('',#110658,4.74975596129105);
#36115=CIRCLE('',#110659,4.72273590800283);
#36116=CIRCLE('',#110660,4.84835211827033);
#36117=CIRCLE('',#110661,3.13054999999999);
#36118=CIRCLE('',#110663,4.74980000000001);
#36119=CIRCLE('',#110664,4.72926310421625);
#36120=CIRCLE('',#110665,4.77210660304378);
#36121=CIRCLE('',#110666,4.74980000000001);
#36122=CIRCLE('',#110667,3.98780000000001);
#36123=CIRCLE('',#110671,2.7496306570156);
#36124=CIRCLE('',#110672,2.7496306570156);
#36125=CIRCLE('',#110673,2.7496306570156);
#36126=CIRCLE('',#110674,2.7496306570156);
#36127=CIRCLE('',#110675,2.7496306570156);
#36128=CIRCLE('',#110676,2.7496306570156);
#36129=CIRCLE('',#110692,40.);
#36130=CIRCLE('',#110693,41.2700000000001);
#36131=CIRCLE('',#110695,40.);
#36132=CIRCLE('',#110696,40.);
#36133=CIRCLE('',#110697,41.2700000000001);
#36134=CIRCLE('',#110699,50.);
#36135=CIRCLE('',#110700,48.4864729374055);
#36136=CIRCLE('',#110702,50.);
#36137=CIRCLE('',#110703,50.);
#36138=CIRCLE('',#110704,48.4864729374054);
#36139=CIRCLE('',#110712,65.0000000000002);
#36140=CIRCLE('',#110713,65.0000000000002);
#36141=CIRCLE('',#110715,56.8750000000002);
#36142=CIRCLE('',#110716,56.875);
#36143=CIRCLE('',#110718,74.8702478255888);
#36144=CIRCLE('',#110719,1.5875);
#36145=CIRCLE('',#110720,76.4577478255888);
#36146=CIRCLE('',#110721,76.4577478255888);
#36147=CIRCLE('',#110723,76.4577478255888);
#36148=CIRCLE('',#110725,66.9885441972308);
#36149=CIRCLE('',#110726,66.9885441972308);
#36150=CIRCLE('',#110728,70.625);
#36151=CIRCLE('',#110729,70.625);
#36152=CIRCLE('',#110731,76.5847478255888);
#36153=CIRCLE('',#110732,76.5847478255888);
#36154=CIRCLE('',#110734,8.4455);
#36155=CIRCLE('',#110735,8.4455);
#36156=CIRCLE('',#110737,8.4455);
#36157=CIRCLE('',#110738,8.4455);
#36158=CIRCLE('',#110740,8.4455);
#36159=CIRCLE('',#110741,8.4455);
#36160=CIRCLE('',#110743,8.4455);
#36161=CIRCLE('',#110744,8.4455);
#36162=CIRCLE('',#110746,7.9375);
#36163=CIRCLE('',#110747,7.9375);
#36164=CIRCLE('',#110749,7.93750000000014);
#36165=CIRCLE('',#110750,7.9375);
#36166=CIRCLE('',#110752,7.93749999999989);
#36167=CIRCLE('',#110753,7.9375);
#36168=CIRCLE('',#110755,7.9375);
#36169=CIRCLE('',#110756,7.9375);
#36170=CIRCLE('',#110758,24.492);
#36171=CIRCLE('',#110759,24.492);
#36172=CIRCLE('',#110762,24.492);
#36173=CIRCLE('',#110763,24.492);
#36174=CIRCLE('',#110766,24.492);
#36175=CIRCLE('',#110767,24.492);
#36176=CIRCLE('',#110770,24.492);
#36177=CIRCLE('',#110771,24.492);
#36178=CIRCLE('',#110774,23.73);
#36179=CIRCLE('',#110775,23.73);
#36180=CIRCLE('',#110776,23.73);
#36181=CIRCLE('',#110777,23.73);
#36182=CIRCLE('',#110783,25.);
#36183=CIRCLE('',#110784,25.);
#36184=CIRCLE('',#110785,25.);
#36185=CIRCLE('',#110786,25.);
#36186=CIRCLE('',#110788,25.);
#36187=CIRCLE('',#110791,25.);
#36188=CIRCLE('',#110794,25.);
#36189=CIRCLE('',#110797,25.);
#36190=CIRCLE('',#110800,0.762);
#36191=CIRCLE('',#110801,0.762);
#36192=CIRCLE('',#110803,0.762);
#36193=CIRCLE('',#110805,0.762);
#36194=CIRCLE('',#110807,0.762);
#36195=CIRCLE('',#110809,0.762);
#36196=CIRCLE('',#110811,0.762);
#36197=CIRCLE('',#110813,0.762);
#36198=CIRCLE('',#110817,66.9885441972308);
#36199=CIRCLE('',#110818,66.9885441972308);
#36200=CIRCLE('',#110820,73.6560441972308);
#36201=CIRCLE('',#110821,73.6560441972308);
#36202=CIRCLE('',#110826,73.6560441972308);
#36203=CIRCLE('',#110830,73.6560441972308);
#36725=VERTEX_POINT('',#167146);
#36726=VERTEX_POINT('',#167148);
#36727=VERTEX_POINT('',#167150);
#36728=VERTEX_POINT('',#167154);
#36729=VERTEX_POINT('',#167155);
#36730=VERTEX_POINT('',#167166);
#36731=VERTEX_POINT('',#167168);
#36732=VERTEX_POINT('',#167181);
#36733=VERTEX_POINT('',#167182);
#36734=VERTEX_POINT('',#167191);
#36735=VERTEX_POINT('',#167193);
#36736=VERTEX_POINT('',#167197);
#36737=VERTEX_POINT('',#167198);
#36738=VERTEX_POINT('',#167200);
#36739=VERTEX_POINT('',#167204);
#36740=VERTEX_POINT('',#167215);
#36741=VERTEX_POINT('',#167221);
#36742=VERTEX_POINT('',#167222);
#36743=VERTEX_POINT('',#167224);
#36744=VERTEX_POINT('',#167228);
#36745=VERTEX_POINT('',#167232);
#36746=VERTEX_POINT('',#167235);
#36747=VERTEX_POINT('',#167236);
#36748=VERTEX_POINT('',#167241);
#36749=VERTEX_POINT('',#167243);
#36750=VERTEX_POINT('',#167247);
#36751=VERTEX_POINT('',#167251);
#36752=VERTEX_POINT('',#167253);
#36753=VERTEX_POINT('',#167266);
#36754=VERTEX_POINT('',#167270);
#36755=VERTEX_POINT('',#167285);
#36756=VERTEX_POINT('',#167289);
#36757=VERTEX_POINT('',#167304);
#36758=VERTEX_POINT('',#167308);
#36759=VERTEX_POINT('',#167323);
#36760=VERTEX_POINT('',#167327);
#36761=VERTEX_POINT('',#167343);
#36762=VERTEX_POINT('',#167345);
#36763=VERTEX_POINT('',#167347);
#36764=VERTEX_POINT('',#167349);
#36765=VERTEX_POINT('',#167353);
#36766=VERTEX_POINT('',#167357);
#36767=VERTEX_POINT('',#167372);
#36768=VERTEX_POINT('',#167376);
#36769=VERTEX_POINT('',#167391);
#36770=VERTEX_POINT('',#167395);
#36771=VERTEX_POINT('',#167410);
#36772=VERTEX_POINT('',#167414);
#36773=VERTEX_POINT('',#167429);
#36774=VERTEX_POINT('',#167433);
#36775=VERTEX_POINT('',#167469);
#36776=VERTEX_POINT('',#167471);
#36777=VERTEX_POINT('',#167475);
#36778=VERTEX_POINT('',#167477);
#36779=VERTEX_POINT('',#167483);
#36780=VERTEX_POINT('',#167485);
#36781=VERTEX_POINT('',#167489);
#36782=VERTEX_POINT('',#167491);
#36783=VERTEX_POINT('',#167497);
#36784=VERTEX_POINT('',#167499);
#36785=VERTEX_POINT('',#167503);
#36786=VERTEX_POINT('',#167505);
#36787=VERTEX_POINT('',#167511);
#36788=VERTEX_POINT('',#167513);
#36789=VERTEX_POINT('',#167517);
#36790=VERTEX_POINT('',#167519);
#36791=VERTEX_POINT('',#167525);
#36792=VERTEX_POINT('',#167526);
#36793=VERTEX_POINT('',#167529);
#36794=VERTEX_POINT('',#167533);
#36795=VERTEX_POINT('',#167535);
#36796=VERTEX_POINT('',#167537);
#36797=VERTEX_POINT('',#167541);
#36798=VERTEX_POINT('',#167545);
#36799=VERTEX_POINT('',#167551);
#36800=VERTEX_POINT('',#167553);
#36801=VERTEX_POINT('',#167555);
#36802=VERTEX_POINT('',#167559);
#36803=VERTEX_POINT('',#167560);
#36804=VERTEX_POINT('',#167563);
#36805=VERTEX_POINT('',#167567);
#36806=VERTEX_POINT('',#167571);
#36807=VERTEX_POINT('',#167577);
#36808=VERTEX_POINT('',#167579);
#36809=VERTEX_POINT('',#167583);
#36810=VERTEX_POINT('',#167585);
#36811=VERTEX_POINT('',#167591);
#36812=VERTEX_POINT('',#167592);
#36813=VERTEX_POINT('',#167594);
#36814=VERTEX_POINT('',#167596);
#36815=VERTEX_POINT('',#167600);
#36816=VERTEX_POINT('',#167601);
#36817=VERTEX_POINT('',#167603);
#36818=VERTEX_POINT('',#167605);
#36819=VERTEX_POINT('',#167609);
#36820=VERTEX_POINT('',#167610);
#36821=VERTEX_POINT('',#167612);
#36822=VERTEX_POINT('',#167614);
#36823=VERTEX_POINT('',#167618);
#36824=VERTEX_POINT('',#167619);
#36825=VERTEX_POINT('',#167621);
#36826=VERTEX_POINT('',#167623);
#36827=VERTEX_POINT('',#167625);
#36828=VERTEX_POINT('',#167629);
#36829=VERTEX_POINT('',#167631);
#36830=VERTEX_POINT('',#167633);
#36831=VERTEX_POINT('',#167637);
#36832=VERTEX_POINT('',#167639);
#36833=VERTEX_POINT('',#167643);
#36834=VERTEX_POINT('',#167645);
#36835=VERTEX_POINT('',#167647);
#36836=VERTEX_POINT('',#167651);
#36837=VERTEX_POINT('',#167653);
#36838=VERTEX_POINT('',#167657);
#36839=VERTEX_POINT('',#167659);
#36840=VERTEX_POINT('',#167665);
#36841=VERTEX_POINT('',#167666);
#36842=VERTEX_POINT('',#167668);
#36843=VERTEX_POINT('',#167712);
#36844=VERTEX_POINT('',#167714);
#36845=VERTEX_POINT('',#167716);
#36846=VERTEX_POINT('',#167718);
#36847=VERTEX_POINT('',#167759);
#36848=VERTEX_POINT('',#167761);
#36849=VERTEX_POINT('',#167805);
#36850=VERTEX_POINT('',#167807);
#36851=VERTEX_POINT('',#167809);
#36852=VERTEX_POINT('',#167811);
#36853=VERTEX_POINT('',#167852);
#36854=VERTEX_POINT('',#167854);
#36855=VERTEX_POINT('',#167898);
#36856=VERTEX_POINT('',#167900);
#36857=VERTEX_POINT('',#167902);
#36858=VERTEX_POINT('',#167904);
#36859=VERTEX_POINT('',#167945);
#36860=VERTEX_POINT('',#167947);
#36861=VERTEX_POINT('',#167991);
#36862=VERTEX_POINT('',#167993);
#36863=VERTEX_POINT('',#167995);
#36864=VERTEX_POINT('',#167997);
#36865=VERTEX_POINT('',#168038);
#36866=VERTEX_POINT('',#168040);
#36867=VERTEX_POINT('',#168084);
#36868=VERTEX_POINT('',#168086);
#36869=VERTEX_POINT('',#168088);
#36870=VERTEX_POINT('',#168090);
#36871=VERTEX_POINT('',#168131);
#36872=VERTEX_POINT('',#168133);
#36873=VERTEX_POINT('',#168177);
#36874=VERTEX_POINT('',#168179);
#36875=VERTEX_POINT('',#168181);
#36876=VERTEX_POINT('',#168183);
#36877=VERTEX_POINT('',#168224);
#36878=VERTEX_POINT('',#168226);
#36879=VERTEX_POINT('',#168270);
#36880=VERTEX_POINT('',#168272);
#36881=VERTEX_POINT('',#168274);
#36882=VERTEX_POINT('',#168276);
#36883=VERTEX_POINT('',#168317);
#36884=VERTEX_POINT('',#168319);
#36885=VERTEX_POINT('',#168363);
#36886=VERTEX_POINT('',#168365);
#36887=VERTEX_POINT('',#168367);
#36888=VERTEX_POINT('',#168369);
#36889=VERTEX_POINT('',#168410);
#36890=VERTEX_POINT('',#168412);
#36891=VERTEX_POINT('',#168456);
#36892=VERTEX_POINT('',#168458);
#36893=VERTEX_POINT('',#168460);
#36894=VERTEX_POINT('',#168462);
#36895=VERTEX_POINT('',#168503);
#36896=VERTEX_POINT('',#168505);
#36897=VERTEX_POINT('',#168549);
#36898=VERTEX_POINT('',#168551);
#36899=VERTEX_POINT('',#168553);
#36900=VERTEX_POINT('',#168555);
#36901=VERTEX_POINT('',#168596);
#36902=VERTEX_POINT('',#168598);
#36903=VERTEX_POINT('',#168642);
#36904=VERTEX_POINT('',#168644);
#36905=VERTEX_POINT('',#168646);
#36906=VERTEX_POINT('',#168648);
#36907=VERTEX_POINT('',#168689);
#36908=VERTEX_POINT('',#168691);
#36909=VERTEX_POINT('',#168735);
#36910=VERTEX_POINT('',#168737);
#36911=VERTEX_POINT('',#168739);
#36912=VERTEX_POINT('',#168741);
#36913=VERTEX_POINT('',#168782);
#36914=VERTEX_POINT('',#168784);
#36915=VERTEX_POINT('',#168828);
#36916=VERTEX_POINT('',#168830);
#36917=VERTEX_POINT('',#168832);
#36918=VERTEX_POINT('',#168834);
#36919=VERTEX_POINT('',#168875);
#36920=VERTEX_POINT('',#168877);
#36921=VERTEX_POINT('',#168921);
#36922=VERTEX_POINT('',#168923);
#36923=VERTEX_POINT('',#168925);
#36924=VERTEX_POINT('',#168927);
#36925=VERTEX_POINT('',#168968);
#36926=VERTEX_POINT('',#168970);
#36927=VERTEX_POINT('',#169014);
#36928=VERTEX_POINT('',#169016);
#36929=VERTEX_POINT('',#169018);
#36930=VERTEX_POINT('',#169020);
#36931=VERTEX_POINT('',#169061);
#36932=VERTEX_POINT('',#169063);
#36933=VERTEX_POINT('',#169107);
#36934=VERTEX_POINT('',#169109);
#36935=VERTEX_POINT('',#169111);
#36936=VERTEX_POINT('',#169113);
#36937=VERTEX_POINT('',#169154);
#36938=VERTEX_POINT('',#169156);
#36939=VERTEX_POINT('',#169200);
#36940=VERTEX_POINT('',#169202);
#36941=VERTEX_POINT('',#169204);
#36942=VERTEX_POINT('',#169206);
#36943=VERTEX_POINT('',#169247);
#36944=VERTEX_POINT('',#169249);
#36945=VERTEX_POINT('',#169293);
#36946=VERTEX_POINT('',#169295);
#36947=VERTEX_POINT('',#169297);
#36948=VERTEX_POINT('',#169299);
#36949=VERTEX_POINT('',#169340);
#36950=VERTEX_POINT('',#169342);
#36951=VERTEX_POINT('',#169386);
#36952=VERTEX_POINT('',#169388);
#36953=VERTEX_POINT('',#169390);
#36954=VERTEX_POINT('',#169392);
#36955=VERTEX_POINT('',#169433);
#36956=VERTEX_POINT('',#169435);
#36957=VERTEX_POINT('',#169479);
#36958=VERTEX_POINT('',#169481);
#36959=VERTEX_POINT('',#169483);
#36960=VERTEX_POINT('',#169485);
#36961=VERTEX_POINT('',#169526);
#36962=VERTEX_POINT('',#169528);
#36963=VERTEX_POINT('',#169572);
#36964=VERTEX_POINT('',#169574);
#36965=VERTEX_POINT('',#169576);
#36966=VERTEX_POINT('',#169578);
#36967=VERTEX_POINT('',#169619);
#36968=VERTEX_POINT('',#169621);
#36969=VERTEX_POINT('',#169665);
#36970=VERTEX_POINT('',#169667);
#36971=VERTEX_POINT('',#169669);
#36972=VERTEX_POINT('',#169671);
#36973=VERTEX_POINT('',#169712);
#36974=VERTEX_POINT('',#169714);
#36975=VERTEX_POINT('',#169758);
#36976=VERTEX_POINT('',#169760);
#36977=VERTEX_POINT('',#169762);
#36978=VERTEX_POINT('',#169764);
#36979=VERTEX_POINT('',#169805);
#36980=VERTEX_POINT('',#169807);
#36981=VERTEX_POINT('',#169851);
#36982=VERTEX_POINT('',#169853);
#36983=VERTEX_POINT('',#169855);
#36984=VERTEX_POINT('',#169857);
#36985=VERTEX_POINT('',#169898);
#36986=VERTEX_POINT('',#169900);
#36987=VERTEX_POINT('',#169944);
#36988=VERTEX_POINT('',#169946);
#36989=VERTEX_POINT('',#169948);
#36990=VERTEX_POINT('',#169950);
#36991=VERTEX_POINT('',#169991);
#36992=VERTEX_POINT('',#169993);
#36993=VERTEX_POINT('',#170037);
#36994=VERTEX_POINT('',#170039);
#36995=VERTEX_POINT('',#170041);
#36996=VERTEX_POINT('',#170043);
#36997=VERTEX_POINT('',#170084);
#36998=VERTEX_POINT('',#170086);
#36999=VERTEX_POINT('',#170130);
#37000=VERTEX_POINT('',#170132);
#37001=VERTEX_POINT('',#170134);
#37002=VERTEX_POINT('',#170136);
#37003=VERTEX_POINT('',#170177);
#37004=VERTEX_POINT('',#170179);
#37005=VERTEX_POINT('',#170223);
#37006=VERTEX_POINT('',#170225);
#37007=VERTEX_POINT('',#170227);
#37008=VERTEX_POINT('',#170229);
#37009=VERTEX_POINT('',#170270);
#37010=VERTEX_POINT('',#170272);
#37011=VERTEX_POINT('',#170316);
#37012=VERTEX_POINT('',#170318);
#37013=VERTEX_POINT('',#170320);
#37014=VERTEX_POINT('',#170322);
#37015=VERTEX_POINT('',#170363);
#37016=VERTEX_POINT('',#170365);
#37017=VERTEX_POINT('',#170409);
#37018=VERTEX_POINT('',#170411);
#37019=VERTEX_POINT('',#170413);
#37020=VERTEX_POINT('',#170456);
#37021=VERTEX_POINT('',#170500);
#37022=VERTEX_POINT('',#170502);
#37023=VERTEX_POINT('',#170504);
#37024=VERTEX_POINT('',#170506);
#37025=VERTEX_POINT('',#170547);
#37026=VERTEX_POINT('',#170549);
#37027=VERTEX_POINT('',#170593);
#37028=VERTEX_POINT('',#170595);
#37029=VERTEX_POINT('',#170597);
#37030=VERTEX_POINT('',#170599);
#37031=VERTEX_POINT('',#170640);
#37032=VERTEX_POINT('',#170642);
#37033=VERTEX_POINT('',#170686);
#37034=VERTEX_POINT('',#170688);
#37035=VERTEX_POINT('',#170690);
#37036=VERTEX_POINT('',#170692);
#37037=VERTEX_POINT('',#170733);
#37038=VERTEX_POINT('',#170735);
#37039=VERTEX_POINT('',#170779);
#37040=VERTEX_POINT('',#170781);
#37041=VERTEX_POINT('',#170783);
#37042=VERTEX_POINT('',#170785);
#37043=VERTEX_POINT('',#170826);
#37044=VERTEX_POINT('',#170828);
#37045=VERTEX_POINT('',#170872);
#37046=VERTEX_POINT('',#170874);
#37047=VERTEX_POINT('',#170876);
#37048=VERTEX_POINT('',#170878);
#37049=VERTEX_POINT('',#170919);
#37050=VERTEX_POINT('',#170921);
#37051=VERTEX_POINT('',#170965);
#37052=VERTEX_POINT('',#170967);
#37053=VERTEX_POINT('',#170969);
#37054=VERTEX_POINT('',#170971);
#37055=VERTEX_POINT('',#171012);
#37056=VERTEX_POINT('',#171014);
#37057=VERTEX_POINT('',#171058);
#37058=VERTEX_POINT('',#171060);
#37059=VERTEX_POINT('',#171062);
#37060=VERTEX_POINT('',#171064);
#37061=VERTEX_POINT('',#171105);
#37062=VERTEX_POINT('',#171107);
#37063=VERTEX_POINT('',#171151);
#37064=VERTEX_POINT('',#171153);
#37065=VERTEX_POINT('',#171155);
#37066=VERTEX_POINT('',#171157);
#37067=VERTEX_POINT('',#171198);
#37068=VERTEX_POINT('',#171200);
#37069=VERTEX_POINT('',#171244);
#37070=VERTEX_POINT('',#171246);
#37071=VERTEX_POINT('',#171248);
#37072=VERTEX_POINT('',#171250);
#37073=VERTEX_POINT('',#171291);
#37074=VERTEX_POINT('',#171293);
#37075=VERTEX_POINT('',#171337);
#37076=VERTEX_POINT('',#171339);
#37077=VERTEX_POINT('',#171341);
#37078=VERTEX_POINT('',#171343);
#37079=VERTEX_POINT('',#171384);
#37080=VERTEX_POINT('',#171386);
#37081=VERTEX_POINT('',#171430);
#37082=VERTEX_POINT('',#171432);
#37083=VERTEX_POINT('',#171434);
#37084=VERTEX_POINT('',#171436);
#37085=VERTEX_POINT('',#171477);
#37086=VERTEX_POINT('',#171479);
#37087=VERTEX_POINT('',#171523);
#37088=VERTEX_POINT('',#171525);
#37089=VERTEX_POINT('',#171527);
#37090=VERTEX_POINT('',#171529);
#37091=VERTEX_POINT('',#171570);
#37092=VERTEX_POINT('',#171572);
#37093=VERTEX_POINT('',#171616);
#37094=VERTEX_POINT('',#171618);
#37095=VERTEX_POINT('',#171620);
#37096=VERTEX_POINT('',#171622);
#37097=VERTEX_POINT('',#171663);
#37098=VERTEX_POINT('',#171665);
#37099=VERTEX_POINT('',#171709);
#37100=VERTEX_POINT('',#171711);
#37101=VERTEX_POINT('',#171713);
#37102=VERTEX_POINT('',#171715);
#37103=VERTEX_POINT('',#171756);
#37104=VERTEX_POINT('',#171758);
#37105=VERTEX_POINT('',#171802);
#37106=VERTEX_POINT('',#171804);
#37107=VERTEX_POINT('',#171806);
#37108=VERTEX_POINT('',#171848);
#37109=VERTEX_POINT('',#171892);
#37110=VERTEX_POINT('',#171894);
#37111=VERTEX_POINT('',#171896);
#37112=VERTEX_POINT('',#171898);
#37113=VERTEX_POINT('',#171939);
#37114=VERTEX_POINT('',#171941);
#37115=VERTEX_POINT('',#171985);
#37116=VERTEX_POINT('',#171987);
#37117=VERTEX_POINT('',#171989);
#37118=VERTEX_POINT('',#171991);
#37119=VERTEX_POINT('',#172032);
#37120=VERTEX_POINT('',#172034);
#37121=VERTEX_POINT('',#172078);
#37122=VERTEX_POINT('',#172080);
#37123=VERTEX_POINT('',#172082);
#37124=VERTEX_POINT('',#172084);
#37125=VERTEX_POINT('',#172125);
#37126=VERTEX_POINT('',#172127);
#37127=VERTEX_POINT('',#172171);
#37128=VERTEX_POINT('',#172173);
#37129=VERTEX_POINT('',#172175);
#37130=VERTEX_POINT('',#172177);
#37131=VERTEX_POINT('',#172218);
#37132=VERTEX_POINT('',#172220);
#37133=VERTEX_POINT('',#172264);
#37134=VERTEX_POINT('',#172266);
#37135=VERTEX_POINT('',#172268);
#37136=VERTEX_POINT('',#172270);
#37137=VERTEX_POINT('',#172311);
#37138=VERTEX_POINT('',#172313);
#37139=VERTEX_POINT('',#172357);
#37140=VERTEX_POINT('',#172359);
#37141=VERTEX_POINT('',#172361);
#37142=VERTEX_POINT('',#172363);
#37143=VERTEX_POINT('',#172404);
#37144=VERTEX_POINT('',#172406);
#37145=VERTEX_POINT('',#172450);
#37146=VERTEX_POINT('',#172452);
#37147=VERTEX_POINT('',#172454);
#37148=VERTEX_POINT('',#172456);
#37149=VERTEX_POINT('',#172497);
#37150=VERTEX_POINT('',#172499);
#37151=VERTEX_POINT('',#172543);
#37152=VERTEX_POINT('',#172545);
#37153=VERTEX_POINT('',#172547);
#37154=VERTEX_POINT('',#172549);
#37155=VERTEX_POINT('',#172590);
#37156=VERTEX_POINT('',#172592);
#37157=VERTEX_POINT('',#172636);
#37158=VERTEX_POINT('',#172638);
#37159=VERTEX_POINT('',#172640);
#37160=VERTEX_POINT('',#172642);
#37161=VERTEX_POINT('',#172683);
#37162=VERTEX_POINT('',#172685);
#37163=VERTEX_POINT('',#172729);
#37164=VERTEX_POINT('',#172731);
#37165=VERTEX_POINT('',#172733);
#37166=VERTEX_POINT('',#172735);
#37167=VERTEX_POINT('',#172776);
#37168=VERTEX_POINT('',#172778);
#37169=VERTEX_POINT('',#172822);
#37170=VERTEX_POINT('',#172824);
#37171=VERTEX_POINT('',#172826);
#37172=VERTEX_POINT('',#172828);
#37173=VERTEX_POINT('',#172869);
#37174=VERTEX_POINT('',#172871);
#37175=VERTEX_POINT('',#172915);
#37176=VERTEX_POINT('',#172917);
#37177=VERTEX_POINT('',#172919);
#37178=VERTEX_POINT('',#172921);
#37179=VERTEX_POINT('',#172962);
#37180=VERTEX_POINT('',#172964);
#37181=VERTEX_POINT('',#173008);
#37182=VERTEX_POINT('',#173010);
#37183=VERTEX_POINT('',#173012);
#37184=VERTEX_POINT('',#173014);
#37185=VERTEX_POINT('',#173055);
#37186=VERTEX_POINT('',#173057);
#37187=VERTEX_POINT('',#173101);
#37188=VERTEX_POINT('',#173103);
#37189=VERTEX_POINT('',#173105);
#37190=VERTEX_POINT('',#173107);
#37191=VERTEX_POINT('',#173148);
#37192=VERTEX_POINT('',#173150);
#37193=VERTEX_POINT('',#173194);
#37194=VERTEX_POINT('',#173196);
#37195=VERTEX_POINT('',#173198);
#37196=VERTEX_POINT('',#173241);
#37197=VERTEX_POINT('',#173279);
#37198=VERTEX_POINT('',#173281);
#37199=VERTEX_POINT('',#173283);
#37200=VERTEX_POINT('',#173285);
#37201=VERTEX_POINT('',#173326);
#37202=VERTEX_POINT('',#173328);
#37203=VERTEX_POINT('',#173366);
#37204=VERTEX_POINT('',#173368);
#37205=VERTEX_POINT('',#173370);
#37206=VERTEX_POINT('',#173372);
#37207=VERTEX_POINT('',#173413);
#37208=VERTEX_POINT('',#173415);
#37209=VERTEX_POINT('',#173453);
#37210=VERTEX_POINT('',#173455);
#37211=VERTEX_POINT('',#173457);
#37212=VERTEX_POINT('',#173459);
#37213=VERTEX_POINT('',#173500);
#37214=VERTEX_POINT('',#173502);
#37215=VERTEX_POINT('',#173540);
#37216=VERTEX_POINT('',#173542);
#37217=VERTEX_POINT('',#173544);
#37218=VERTEX_POINT('',#173546);
#37219=VERTEX_POINT('',#173587);
#37220=VERTEX_POINT('',#173589);
#37221=VERTEX_POINT('',#173627);
#37222=VERTEX_POINT('',#173629);
#37223=VERTEX_POINT('',#173631);
#37224=VERTEX_POINT('',#173633);
#37225=VERTEX_POINT('',#173674);
#37226=VERTEX_POINT('',#173676);
#37227=VERTEX_POINT('',#173714);
#37228=VERTEX_POINT('',#173716);
#37229=VERTEX_POINT('',#173718);
#37230=VERTEX_POINT('',#173720);
#37231=VERTEX_POINT('',#173761);
#37232=VERTEX_POINT('',#173763);
#37233=VERTEX_POINT('',#173801);
#37234=VERTEX_POINT('',#173803);
#37235=VERTEX_POINT('',#173805);
#37236=VERTEX_POINT('',#173807);
#37237=VERTEX_POINT('',#173848);
#37238=VERTEX_POINT('',#173850);
#37239=VERTEX_POINT('',#173888);
#37240=VERTEX_POINT('',#173890);
#37241=VERTEX_POINT('',#173892);
#37242=VERTEX_POINT('',#173894);
#37243=VERTEX_POINT('',#173935);
#37244=VERTEX_POINT('',#173937);
#37245=VERTEX_POINT('',#173975);
#37246=VERTEX_POINT('',#173977);
#37247=VERTEX_POINT('',#173979);
#37248=VERTEX_POINT('',#173981);
#37249=VERTEX_POINT('',#174022);
#37250=VERTEX_POINT('',#174024);
#37251=VERTEX_POINT('',#174062);
#37252=VERTEX_POINT('',#174064);
#37253=VERTEX_POINT('',#174066);
#37254=VERTEX_POINT('',#174068);
#37255=VERTEX_POINT('',#174109);
#37256=VERTEX_POINT('',#174111);
#37257=VERTEX_POINT('',#174149);
#37258=VERTEX_POINT('',#174151);
#37259=VERTEX_POINT('',#174153);
#37260=VERTEX_POINT('',#174155);
#37261=VERTEX_POINT('',#174196);
#37262=VERTEX_POINT('',#174198);
#37263=VERTEX_POINT('',#174236);
#37264=VERTEX_POINT('',#174238);
#37265=VERTEX_POINT('',#174240);
#37266=VERTEX_POINT('',#174242);
#37267=VERTEX_POINT('',#174283);
#37268=VERTEX_POINT('',#174285);
#37269=VERTEX_POINT('',#174323);
#37270=VERTEX_POINT('',#174325);
#37271=VERTEX_POINT('',#174327);
#37272=VERTEX_POINT('',#174329);
#37273=VERTEX_POINT('',#174370);
#37274=VERTEX_POINT('',#174372);
#37275=VERTEX_POINT('',#174410);
#37276=VERTEX_POINT('',#174412);
#37277=VERTEX_POINT('',#174414);
#37278=VERTEX_POINT('',#174416);
#37279=VERTEX_POINT('',#174457);
#37280=VERTEX_POINT('',#174459);
#37281=VERTEX_POINT('',#174497);
#37282=VERTEX_POINT('',#174499);
#37283=VERTEX_POINT('',#174501);
#37284=VERTEX_POINT('',#174503);
#37285=VERTEX_POINT('',#174544);
#37286=VERTEX_POINT('',#174546);
#37287=VERTEX_POINT('',#174584);
#37288=VERTEX_POINT('',#174586);
#37289=VERTEX_POINT('',#174588);
#37290=VERTEX_POINT('',#174590);
#37291=VERTEX_POINT('',#174631);
#37292=VERTEX_POINT('',#174633);
#37293=VERTEX_POINT('',#174671);
#37294=VERTEX_POINT('',#174673);
#37295=VERTEX_POINT('',#174675);
#37296=VERTEX_POINT('',#174677);
#37297=VERTEX_POINT('',#174718);
#37298=VERTEX_POINT('',#174720);
#37299=VERTEX_POINT('',#174758);
#37300=VERTEX_POINT('',#174760);
#37301=VERTEX_POINT('',#174762);
#37302=VERTEX_POINT('',#174764);
#37303=VERTEX_POINT('',#174805);
#37304=VERTEX_POINT('',#174807);
#37305=VERTEX_POINT('',#174845);
#37306=VERTEX_POINT('',#174847);
#37307=VERTEX_POINT('',#174849);
#37308=VERTEX_POINT('',#174851);
#37309=VERTEX_POINT('',#174892);
#37310=VERTEX_POINT('',#174894);
#37311=VERTEX_POINT('',#174932);
#37312=VERTEX_POINT('',#174934);
#37313=VERTEX_POINT('',#174936);
#37314=VERTEX_POINT('',#174938);
#37315=VERTEX_POINT('',#174979);
#37316=VERTEX_POINT('',#174981);
#37317=VERTEX_POINT('',#175019);
#37318=VERTEX_POINT('',#175021);
#37319=VERTEX_POINT('',#175023);
#37320=VERTEX_POINT('',#175025);
#37321=VERTEX_POINT('',#175066);
#37322=VERTEX_POINT('',#175068);
#37323=VERTEX_POINT('',#175106);
#37324=VERTEX_POINT('',#175108);
#37325=VERTEX_POINT('',#175110);
#37326=VERTEX_POINT('',#175112);
#37327=VERTEX_POINT('',#175153);
#37328=VERTEX_POINT('',#175155);
#37329=VERTEX_POINT('',#175193);
#37330=VERTEX_POINT('',#175195);
#37331=VERTEX_POINT('',#175197);
#37332=VERTEX_POINT('',#175199);
#37333=VERTEX_POINT('',#175240);
#37334=VERTEX_POINT('',#175242);
#37335=VERTEX_POINT('',#175280);
#37336=VERTEX_POINT('',#175282);
#37337=VERTEX_POINT('',#175284);
#37338=VERTEX_POINT('',#175286);
#37339=VERTEX_POINT('',#175327);
#37340=VERTEX_POINT('',#175329);
#37341=VERTEX_POINT('',#175367);
#37342=VERTEX_POINT('',#175369);
#37343=VERTEX_POINT('',#175371);
#37344=VERTEX_POINT('',#175373);
#37345=VERTEX_POINT('',#175414);
#37346=VERTEX_POINT('',#175416);
#37347=VERTEX_POINT('',#175454);
#37348=VERTEX_POINT('',#175456);
#37349=VERTEX_POINT('',#175458);
#37350=VERTEX_POINT('',#175460);
#37351=VERTEX_POINT('',#175501);
#37352=VERTEX_POINT('',#175503);
#37353=VERTEX_POINT('',#175541);
#37354=VERTEX_POINT('',#175543);
#37355=VERTEX_POINT('',#175545);
#37356=VERTEX_POINT('',#175547);
#37357=VERTEX_POINT('',#175588);
#37358=VERTEX_POINT('',#175590);
#37359=VERTEX_POINT('',#175628);
#37360=VERTEX_POINT('',#175630);
#37361=VERTEX_POINT('',#175632);
#37362=VERTEX_POINT('',#175634);
#37363=VERTEX_POINT('',#175675);
#37364=VERTEX_POINT('',#175677);
#37365=VERTEX_POINT('',#175715);
#37366=VERTEX_POINT('',#175717);
#37367=VERTEX_POINT('',#175719);
#37368=VERTEX_POINT('',#175721);
#37369=VERTEX_POINT('',#175762);
#37370=VERTEX_POINT('',#175764);
#37371=VERTEX_POINT('',#175802);
#37372=VERTEX_POINT('',#175804);
#37373=VERTEX_POINT('',#175806);
#37374=VERTEX_POINT('',#175808);
#37375=VERTEX_POINT('',#175849);
#37376=VERTEX_POINT('',#175852);
#37377=VERTEX_POINT('',#175854);
#37378=VERTEX_POINT('',#175892);
#37379=VERTEX_POINT('',#175894);
#37380=VERTEX_POINT('',#175896);
#37381=VERTEX_POINT('',#175898);
#37382=VERTEX_POINT('',#175939);
#37383=VERTEX_POINT('',#175941);
#37384=VERTEX_POINT('',#175979);
#37385=VERTEX_POINT('',#175981);
#37386=VERTEX_POINT('',#175983);
#37387=VERTEX_POINT('',#175985);
#37388=VERTEX_POINT('',#176026);
#37389=VERTEX_POINT('',#176028);
#37390=VERTEX_POINT('',#176066);
#37391=VERTEX_POINT('',#176068);
#37392=VERTEX_POINT('',#176070);
#37393=VERTEX_POINT('',#176072);
#37394=VERTEX_POINT('',#176113);
#37395=VERTEX_POINT('',#176115);
#37396=VERTEX_POINT('',#176153);
#37397=VERTEX_POINT('',#176155);
#37398=VERTEX_POINT('',#176157);
#37399=VERTEX_POINT('',#176159);
#37400=VERTEX_POINT('',#176200);
#37401=VERTEX_POINT('',#176202);
#37402=VERTEX_POINT('',#176240);
#37403=VERTEX_POINT('',#176242);
#37404=VERTEX_POINT('',#176244);
#37405=VERTEX_POINT('',#176246);
#37406=VERTEX_POINT('',#176287);
#37407=VERTEX_POINT('',#176289);
#37408=VERTEX_POINT('',#176327);
#37409=VERTEX_POINT('',#176329);
#37410=VERTEX_POINT('',#176331);
#37411=VERTEX_POINT('',#176333);
#37412=VERTEX_POINT('',#176374);
#37413=VERTEX_POINT('',#176376);
#37414=VERTEX_POINT('',#176414);
#37415=VERTEX_POINT('',#176416);
#37416=VERTEX_POINT('',#176418);
#37417=VERTEX_POINT('',#176420);
#37418=VERTEX_POINT('',#176461);
#37419=VERTEX_POINT('',#176463);
#37420=VERTEX_POINT('',#176501);
#37421=VERTEX_POINT('',#176503);
#37422=VERTEX_POINT('',#176505);
#37423=VERTEX_POINT('',#176507);
#37424=VERTEX_POINT('',#176548);
#37425=VERTEX_POINT('',#176550);
#37426=VERTEX_POINT('',#176588);
#37427=VERTEX_POINT('',#176590);
#37428=VERTEX_POINT('',#176592);
#37429=VERTEX_POINT('',#176594);
#37430=VERTEX_POINT('',#176635);
#37431=VERTEX_POINT('',#176637);
#37432=VERTEX_POINT('',#176675);
#37433=VERTEX_POINT('',#176677);
#37434=VERTEX_POINT('',#176679);
#37435=VERTEX_POINT('',#176681);
#37436=VERTEX_POINT('',#176722);
#37437=VERTEX_POINT('',#176724);
#37438=VERTEX_POINT('',#176762);
#37439=VERTEX_POINT('',#176764);
#37440=VERTEX_POINT('',#176766);
#37441=VERTEX_POINT('',#176768);
#37442=VERTEX_POINT('',#176809);
#37443=VERTEX_POINT('',#176811);
#37444=VERTEX_POINT('',#176849);
#37445=VERTEX_POINT('',#176851);
#37446=VERTEX_POINT('',#176853);
#37447=VERTEX_POINT('',#176855);
#37448=VERTEX_POINT('',#176896);
#37449=VERTEX_POINT('',#176898);
#37450=VERTEX_POINT('',#176936);
#37451=VERTEX_POINT('',#176938);
#37452=VERTEX_POINT('',#176940);
#37453=VERTEX_POINT('',#176942);
#37454=VERTEX_POINT('',#176983);
#37455=VERTEX_POINT('',#176985);
#37456=VERTEX_POINT('',#177023);
#37457=VERTEX_POINT('',#177025);
#37458=VERTEX_POINT('',#177027);
#37459=VERTEX_POINT('',#177029);
#37460=VERTEX_POINT('',#177070);
#37461=VERTEX_POINT('',#177072);
#37462=VERTEX_POINT('',#177110);
#37463=VERTEX_POINT('',#177112);
#37464=VERTEX_POINT('',#177114);
#37465=VERTEX_POINT('',#177156);
#37466=VERTEX_POINT('',#177194);
#37467=VERTEX_POINT('',#177196);
#37468=VERTEX_POINT('',#177198);
#37469=VERTEX_POINT('',#177200);
#37470=VERTEX_POINT('',#177241);
#37471=VERTEX_POINT('',#177243);
#37472=VERTEX_POINT('',#177281);
#37473=VERTEX_POINT('',#177283);
#37474=VERTEX_POINT('',#177285);
#37475=VERTEX_POINT('',#177287);
#37476=VERTEX_POINT('',#177328);
#37477=VERTEX_POINT('',#177330);
#37478=VERTEX_POINT('',#177368);
#37479=VERTEX_POINT('',#177370);
#37480=VERTEX_POINT('',#177372);
#37481=VERTEX_POINT('',#177374);
#37482=VERTEX_POINT('',#177415);
#37483=VERTEX_POINT('',#177417);
#37484=VERTEX_POINT('',#177455);
#37485=VERTEX_POINT('',#177457);
#37486=VERTEX_POINT('',#177459);
#37487=VERTEX_POINT('',#177461);
#37488=VERTEX_POINT('',#177502);
#37489=VERTEX_POINT('',#177504);
#37490=VERTEX_POINT('',#177542);
#37491=VERTEX_POINT('',#177544);
#37492=VERTEX_POINT('',#177546);
#37493=VERTEX_POINT('',#177548);
#37494=VERTEX_POINT('',#177589);
#37495=VERTEX_POINT('',#177591);
#37496=VERTEX_POINT('',#177629);
#37497=VERTEX_POINT('',#177631);
#37498=VERTEX_POINT('',#177633);
#37499=VERTEX_POINT('',#177635);
#37500=VERTEX_POINT('',#177676);
#37501=VERTEX_POINT('',#177678);
#37502=VERTEX_POINT('',#177716);
#37503=VERTEX_POINT('',#177718);
#37504=VERTEX_POINT('',#177720);
#37505=VERTEX_POINT('',#177722);
#37506=VERTEX_POINT('',#177763);
#37507=VERTEX_POINT('',#177765);
#37508=VERTEX_POINT('',#177803);
#37509=VERTEX_POINT('',#177805);
#37510=VERTEX_POINT('',#177807);
#37511=VERTEX_POINT('',#177809);
#37512=VERTEX_POINT('',#177850);
#37513=VERTEX_POINT('',#177852);
#37514=VERTEX_POINT('',#177890);
#37515=VERTEX_POINT('',#177892);
#37516=VERTEX_POINT('',#177894);
#37517=VERTEX_POINT('',#177896);
#37518=VERTEX_POINT('',#177937);
#37519=VERTEX_POINT('',#177939);
#37520=VERTEX_POINT('',#177977);
#37521=VERTEX_POINT('',#177979);
#37522=VERTEX_POINT('',#177981);
#37523=VERTEX_POINT('',#177983);
#37524=VERTEX_POINT('',#178024);
#37525=VERTEX_POINT('',#178026);
#37526=VERTEX_POINT('',#178064);
#37527=VERTEX_POINT('',#178066);
#37528=VERTEX_POINT('',#178068);
#37529=VERTEX_POINT('',#178070);
#37530=VERTEX_POINT('',#178111);
#37531=VERTEX_POINT('',#178113);
#37532=VERTEX_POINT('',#178151);
#37533=VERTEX_POINT('',#178153);
#37534=VERTEX_POINT('',#178155);
#37535=VERTEX_POINT('',#178157);
#37536=VERTEX_POINT('',#178198);
#37537=VERTEX_POINT('',#178200);
#37538=VERTEX_POINT('',#178238);
#37539=VERTEX_POINT('',#178240);
#37540=VERTEX_POINT('',#178242);
#37541=VERTEX_POINT('',#178244);
#37542=VERTEX_POINT('',#178285);
#37543=VERTEX_POINT('',#178287);
#37544=VERTEX_POINT('',#178325);
#37545=VERTEX_POINT('',#178327);
#37546=VERTEX_POINT('',#178329);
#37547=VERTEX_POINT('',#178331);
#37548=VERTEX_POINT('',#178372);
#37549=VERTEX_POINT('',#178374);
#37550=VERTEX_POINT('',#178412);
#37551=VERTEX_POINT('',#178414);
#37552=VERTEX_POINT('',#178416);
#37553=VERTEX_POINT('',#178459);
#37554=VERTEX_POINT('',#178460);
#37555=VERTEX_POINT('',#178465);
#37556=VERTEX_POINT('',#178469);
#37557=VERTEX_POINT('',#178470);
#37558=VERTEX_POINT('',#178472);
#37559=VERTEX_POINT('',#178474);
#37560=VERTEX_POINT('',#178476);
#37561=VERTEX_POINT('',#178478);
#37562=VERTEX_POINT('',#178482);
#37563=VERTEX_POINT('',#178483);
#37564=VERTEX_POINT('',#178488);
#37565=VERTEX_POINT('',#178489);
#37566=VERTEX_POINT('',#178491);
#37567=VERTEX_POINT('',#178493);
#37568=VERTEX_POINT('',#178497);
#37569=VERTEX_POINT('',#178498);
#37570=VERTEX_POINT('',#178500);
#37571=VERTEX_POINT('',#178502);
#37572=VERTEX_POINT('',#178504);
#37573=VERTEX_POINT('',#178506);
#37574=VERTEX_POINT('',#178510);
#37575=VERTEX_POINT('',#178511);
#37576=VERTEX_POINT('',#178528);
#37577=VERTEX_POINT('',#178529);
#37578=VERTEX_POINT('',#178531);
#37579=VERTEX_POINT('',#178533);
#37580=VERTEX_POINT('',#178535);
#37581=VERTEX_POINT('',#178537);
#37582=VERTEX_POINT('',#178541);
#37583=VERTEX_POINT('',#178543);
#37584=VERTEX_POINT('',#178547);
#37585=VERTEX_POINT('',#178548);
#37586=VERTEX_POINT('',#178550);
#37587=VERTEX_POINT('',#178552);
#37588=VERTEX_POINT('',#178556);
#37589=VERTEX_POINT('',#178557);
#37590=VERTEX_POINT('',#178559);
#37591=VERTEX_POINT('',#178561);
#37592=VERTEX_POINT('',#178563);
#37593=VERTEX_POINT('',#178565);
#37594=VERTEX_POINT('',#178569);
#37595=VERTEX_POINT('',#178571);
#37596=VERTEX_POINT('',#178587);
#37597=VERTEX_POINT('',#178588);
#37598=VERTEX_POINT('',#178590);
#37599=VERTEX_POINT('',#178592);
#37600=VERTEX_POINT('',#178594);
#37601=VERTEX_POINT('',#178596);
#37602=VERTEX_POINT('',#178600);
#37603=VERTEX_POINT('',#178602);
#37604=VERTEX_POINT('',#178606);
#37605=VERTEX_POINT('',#178607);
#37606=VERTEX_POINT('',#178609);
#37607=VERTEX_POINT('',#178611);
#37608=VERTEX_POINT('',#178615);
#37609=VERTEX_POINT('',#178616);
#37610=VERTEX_POINT('',#178618);
#37611=VERTEX_POINT('',#178620);
#37612=VERTEX_POINT('',#178622);
#37613=VERTEX_POINT('',#178624);
#37614=VERTEX_POINT('',#178628);
#37615=VERTEX_POINT('',#178630);
#37616=VERTEX_POINT('',#178646);
#37617=VERTEX_POINT('',#178647);
#37618=VERTEX_POINT('',#178649);
#37619=VERTEX_POINT('',#178651);
#37620=VERTEX_POINT('',#178653);
#37621=VERTEX_POINT('',#178655);
#37622=VERTEX_POINT('',#178659);
#37623=VERTEX_POINT('',#178661);
#37624=VERTEX_POINT('',#178665);
#37625=VERTEX_POINT('',#178666);
#37626=VERTEX_POINT('',#178668);
#37627=VERTEX_POINT('',#178670);
#37628=VERTEX_POINT('',#178674);
#37629=VERTEX_POINT('',#178675);
#37630=VERTEX_POINT('',#178677);
#37631=VERTEX_POINT('',#178679);
#37632=VERTEX_POINT('',#178681);
#37633=VERTEX_POINT('',#178683);
#37634=VERTEX_POINT('',#178687);
#37635=VERTEX_POINT('',#178689);
#37636=VERTEX_POINT('',#178705);
#37637=VERTEX_POINT('',#178706);
#37638=VERTEX_POINT('',#178708);
#37639=VERTEX_POINT('',#178710);
#37640=VERTEX_POINT('',#178712);
#37641=VERTEX_POINT('',#178714);
#37642=VERTEX_POINT('',#178718);
#37643=VERTEX_POINT('',#178720);
#37644=VERTEX_POINT('',#178724);
#37645=VERTEX_POINT('',#178725);
#37646=VERTEX_POINT('',#178727);
#37647=VERTEX_POINT('',#178729);
#37648=VERTEX_POINT('',#178733);
#37649=VERTEX_POINT('',#178734);
#37650=VERTEX_POINT('',#178736);
#37651=VERTEX_POINT('',#178738);
#37652=VERTEX_POINT('',#178740);
#37653=VERTEX_POINT('',#178742);
#37654=VERTEX_POINT('',#178746);
#37655=VERTEX_POINT('',#178748);
#37656=VERTEX_POINT('',#178764);
#37657=VERTEX_POINT('',#178765);
#37658=VERTEX_POINT('',#178767);
#37659=VERTEX_POINT('',#178769);
#37660=VERTEX_POINT('',#178771);
#37661=VERTEX_POINT('',#178773);
#37662=VERTEX_POINT('',#178777);
#37663=VERTEX_POINT('',#178779);
#37664=VERTEX_POINT('',#178783);
#37665=VERTEX_POINT('',#178784);
#37666=VERTEX_POINT('',#178786);
#37667=VERTEX_POINT('',#178788);
#37668=VERTEX_POINT('',#178792);
#37669=VERTEX_POINT('',#178793);
#37670=VERTEX_POINT('',#178795);
#37671=VERTEX_POINT('',#178797);
#37672=VERTEX_POINT('',#178799);
#37673=VERTEX_POINT('',#178801);
#37674=VERTEX_POINT('',#178805);
#37675=VERTEX_POINT('',#178807);
#37676=VERTEX_POINT('',#178823);
#37677=VERTEX_POINT('',#178824);
#37678=VERTEX_POINT('',#178826);
#37679=VERTEX_POINT('',#178828);
#37680=VERTEX_POINT('',#178830);
#37681=VERTEX_POINT('',#178832);
#37682=VERTEX_POINT('',#178836);
#37683=VERTEX_POINT('',#178838);
#37684=VERTEX_POINT('',#178842);
#37685=VERTEX_POINT('',#178843);
#37686=VERTEX_POINT('',#178845);
#37687=VERTEX_POINT('',#178847);
#37688=VERTEX_POINT('',#178851);
#37689=VERTEX_POINT('',#178852);
#37690=VERTEX_POINT('',#178854);
#37691=VERTEX_POINT('',#178856);
#37692=VERTEX_POINT('',#178858);
#37693=VERTEX_POINT('',#178860);
#37694=VERTEX_POINT('',#178864);
#37695=VERTEX_POINT('',#178866);
#37696=VERTEX_POINT('',#178882);
#37697=VERTEX_POINT('',#178883);
#37698=VERTEX_POINT('',#178885);
#37699=VERTEX_POINT('',#178887);
#37700=VERTEX_POINT('',#178889);
#37701=VERTEX_POINT('',#178891);
#37702=VERTEX_POINT('',#178895);
#37703=VERTEX_POINT('',#178897);
#37704=VERTEX_POINT('',#178901);
#37705=VERTEX_POINT('',#178902);
#37706=VERTEX_POINT('',#178904);
#37707=VERTEX_POINT('',#178906);
#37708=VERTEX_POINT('',#178910);
#37709=VERTEX_POINT('',#178911);
#37710=VERTEX_POINT('',#178913);
#37711=VERTEX_POINT('',#178915);
#37712=VERTEX_POINT('',#178917);
#37713=VERTEX_POINT('',#178919);
#37714=VERTEX_POINT('',#178923);
#37715=VERTEX_POINT('',#178925);
#37716=VERTEX_POINT('',#178941);
#37717=VERTEX_POINT('',#178942);
#37718=VERTEX_POINT('',#178944);
#37719=VERTEX_POINT('',#178946);
#37720=VERTEX_POINT('',#178948);
#37721=VERTEX_POINT('',#178950);
#37722=VERTEX_POINT('',#178954);
#37723=VERTEX_POINT('',#178956);
#37724=VERTEX_POINT('',#178960);
#37725=VERTEX_POINT('',#178961);
#37726=VERTEX_POINT('',#178963);
#37727=VERTEX_POINT('',#178965);
#37728=VERTEX_POINT('',#178969);
#37729=VERTEX_POINT('',#178970);
#37730=VERTEX_POINT('',#178972);
#37731=VERTEX_POINT('',#178974);
#37732=VERTEX_POINT('',#178976);
#37733=VERTEX_POINT('',#178978);
#37734=VERTEX_POINT('',#178982);
#37735=VERTEX_POINT('',#178984);
#37736=VERTEX_POINT('',#179000);
#37737=VERTEX_POINT('',#179001);
#37738=VERTEX_POINT('',#179003);
#37739=VERTEX_POINT('',#179005);
#37740=VERTEX_POINT('',#179007);
#37741=VERTEX_POINT('',#179009);
#37742=VERTEX_POINT('',#179013);
#37743=VERTEX_POINT('',#179015);
#37744=VERTEX_POINT('',#179019);
#37745=VERTEX_POINT('',#179020);
#37746=VERTEX_POINT('',#179022);
#37747=VERTEX_POINT('',#179024);
#37748=VERTEX_POINT('',#179028);
#37749=VERTEX_POINT('',#179029);
#37750=VERTEX_POINT('',#179031);
#37751=VERTEX_POINT('',#179033);
#37752=VERTEX_POINT('',#179035);
#37753=VERTEX_POINT('',#179037);
#37754=VERTEX_POINT('',#179041);
#37755=VERTEX_POINT('',#179043);
#37756=VERTEX_POINT('',#179059);
#37757=VERTEX_POINT('',#179060);
#37758=VERTEX_POINT('',#179062);
#37759=VERTEX_POINT('',#179064);
#37760=VERTEX_POINT('',#179066);
#37761=VERTEX_POINT('',#179068);
#37762=VERTEX_POINT('',#179072);
#37763=VERTEX_POINT('',#179074);
#37764=VERTEX_POINT('',#179078);
#37765=VERTEX_POINT('',#179079);
#37766=VERTEX_POINT('',#179081);
#37767=VERTEX_POINT('',#179083);
#37768=VERTEX_POINT('',#179087);
#37769=VERTEX_POINT('',#179088);
#37770=VERTEX_POINT('',#179090);
#37771=VERTEX_POINT('',#179092);
#37772=VERTEX_POINT('',#179094);
#37773=VERTEX_POINT('',#179096);
#37774=VERTEX_POINT('',#179100);
#37775=VERTEX_POINT('',#179102);
#37776=VERTEX_POINT('',#179118);
#37777=VERTEX_POINT('',#179119);
#37778=VERTEX_POINT('',#179121);
#37779=VERTEX_POINT('',#179123);
#37780=VERTEX_POINT('',#179125);
#37781=VERTEX_POINT('',#179127);
#37782=VERTEX_POINT('',#179131);
#37783=VERTEX_POINT('',#179133);
#37784=VERTEX_POINT('',#179137);
#37785=VERTEX_POINT('',#179138);
#37786=VERTEX_POINT('',#179140);
#37787=VERTEX_POINT('',#179142);
#37788=VERTEX_POINT('',#179146);
#37789=VERTEX_POINT('',#179147);
#37790=VERTEX_POINT('',#179149);
#37791=VERTEX_POINT('',#179151);
#37792=VERTEX_POINT('',#179153);
#37793=VERTEX_POINT('',#179155);
#37794=VERTEX_POINT('',#179159);
#37795=VERTEX_POINT('',#179161);
#37796=VERTEX_POINT('',#179177);
#37797=VERTEX_POINT('',#179178);
#37798=VERTEX_POINT('',#179180);
#37799=VERTEX_POINT('',#179182);
#37800=VERTEX_POINT('',#179184);
#37801=VERTEX_POINT('',#179186);
#37802=VERTEX_POINT('',#179190);
#37803=VERTEX_POINT('',#179192);
#37804=VERTEX_POINT('',#179196);
#37805=VERTEX_POINT('',#179197);
#37806=VERTEX_POINT('',#179199);
#37807=VERTEX_POINT('',#179201);
#37808=VERTEX_POINT('',#179205);
#37809=VERTEX_POINT('',#179206);
#37810=VERTEX_POINT('',#179208);
#37811=VERTEX_POINT('',#179210);
#37812=VERTEX_POINT('',#179212);
#37813=VERTEX_POINT('',#179214);
#37814=VERTEX_POINT('',#179218);
#37815=VERTEX_POINT('',#179220);
#37816=VERTEX_POINT('',#179236);
#37817=VERTEX_POINT('',#179237);
#37818=VERTEX_POINT('',#179239);
#37819=VERTEX_POINT('',#179241);
#37820=VERTEX_POINT('',#179243);
#37821=VERTEX_POINT('',#179245);
#37822=VERTEX_POINT('',#179249);
#37823=VERTEX_POINT('',#179251);
#37824=VERTEX_POINT('',#179255);
#37825=VERTEX_POINT('',#179256);
#37826=VERTEX_POINT('',#179258);
#37827=VERTEX_POINT('',#179260);
#37828=VERTEX_POINT('',#179264);
#37829=VERTEX_POINT('',#179265);
#37830=VERTEX_POINT('',#179267);
#37831=VERTEX_POINT('',#179269);
#37832=VERTEX_POINT('',#179271);
#37833=VERTEX_POINT('',#179273);
#37834=VERTEX_POINT('',#179277);
#37835=VERTEX_POINT('',#179279);
#37836=VERTEX_POINT('',#179295);
#37837=VERTEX_POINT('',#179296);
#37838=VERTEX_POINT('',#179298);
#37839=VERTEX_POINT('',#179300);
#37840=VERTEX_POINT('',#179302);
#37841=VERTEX_POINT('',#179304);
#37842=VERTEX_POINT('',#179308);
#37843=VERTEX_POINT('',#179310);
#37844=VERTEX_POINT('',#179314);
#37845=VERTEX_POINT('',#179315);
#37846=VERTEX_POINT('',#179317);
#37847=VERTEX_POINT('',#179319);
#37848=VERTEX_POINT('',#179323);
#37849=VERTEX_POINT('',#179324);
#37850=VERTEX_POINT('',#179326);
#37851=VERTEX_POINT('',#179328);
#37852=VERTEX_POINT('',#179330);
#37853=VERTEX_POINT('',#179332);
#37854=VERTEX_POINT('',#179336);
#37855=VERTEX_POINT('',#179338);
#37856=VERTEX_POINT('',#179354);
#37857=VERTEX_POINT('',#179355);
#37858=VERTEX_POINT('',#179357);
#37859=VERTEX_POINT('',#179359);
#37860=VERTEX_POINT('',#179361);
#37861=VERTEX_POINT('',#179363);
#37862=VERTEX_POINT('',#179367);
#37863=VERTEX_POINT('',#179369);
#37864=VERTEX_POINT('',#179373);
#37865=VERTEX_POINT('',#179374);
#37866=VERTEX_POINT('',#179376);
#37867=VERTEX_POINT('',#179378);
#37868=VERTEX_POINT('',#179382);
#37869=VERTEX_POINT('',#179383);
#37870=VERTEX_POINT('',#179385);
#37871=VERTEX_POINT('',#179387);
#37872=VERTEX_POINT('',#179389);
#37873=VERTEX_POINT('',#179391);
#37874=VERTEX_POINT('',#179395);
#37875=VERTEX_POINT('',#179397);
#37876=VERTEX_POINT('',#179413);
#37877=VERTEX_POINT('',#179414);
#37878=VERTEX_POINT('',#179416);
#37879=VERTEX_POINT('',#179418);
#37880=VERTEX_POINT('',#179420);
#37881=VERTEX_POINT('',#179422);
#37882=VERTEX_POINT('',#179426);
#37883=VERTEX_POINT('',#179428);
#37884=VERTEX_POINT('',#179432);
#37885=VERTEX_POINT('',#179433);
#37886=VERTEX_POINT('',#179435);
#37887=VERTEX_POINT('',#179437);
#37888=VERTEX_POINT('',#179441);
#37889=VERTEX_POINT('',#179442);
#37890=VERTEX_POINT('',#179444);
#37891=VERTEX_POINT('',#179446);
#37892=VERTEX_POINT('',#179448);
#37893=VERTEX_POINT('',#179450);
#37894=VERTEX_POINT('',#179454);
#37895=VERTEX_POINT('',#179456);
#37896=VERTEX_POINT('',#179472);
#37897=VERTEX_POINT('',#179473);
#37898=VERTEX_POINT('',#179475);
#37899=VERTEX_POINT('',#179477);
#37900=VERTEX_POINT('',#179479);
#37901=VERTEX_POINT('',#179481);
#37902=VERTEX_POINT('',#179485);
#37903=VERTEX_POINT('',#179487);
#37904=VERTEX_POINT('',#179491);
#37905=VERTEX_POINT('',#179492);
#37906=VERTEX_POINT('',#179494);
#37907=VERTEX_POINT('',#179496);
#37908=VERTEX_POINT('',#179500);
#37909=VERTEX_POINT('',#179501);
#37910=VERTEX_POINT('',#179503);
#37911=VERTEX_POINT('',#179505);
#37912=VERTEX_POINT('',#179507);
#37913=VERTEX_POINT('',#179509);
#37914=VERTEX_POINT('',#179513);
#37915=VERTEX_POINT('',#179515);
#37916=VERTEX_POINT('',#179531);
#37917=VERTEX_POINT('',#179532);
#37918=VERTEX_POINT('',#179534);
#37919=VERTEX_POINT('',#179536);
#37920=VERTEX_POINT('',#179538);
#37921=VERTEX_POINT('',#179540);
#37922=VERTEX_POINT('',#179544);
#37923=VERTEX_POINT('',#179546);
#37924=VERTEX_POINT('',#179550);
#37925=VERTEX_POINT('',#179551);
#37926=VERTEX_POINT('',#179553);
#37927=VERTEX_POINT('',#179555);
#37928=VERTEX_POINT('',#179559);
#37929=VERTEX_POINT('',#179560);
#37930=VERTEX_POINT('',#179562);
#37931=VERTEX_POINT('',#179564);
#37932=VERTEX_POINT('',#179566);
#37933=VERTEX_POINT('',#179568);
#37934=VERTEX_POINT('',#179572);
#37935=VERTEX_POINT('',#179574);
#37936=VERTEX_POINT('',#179590);
#37937=VERTEX_POINT('',#179591);
#37938=VERTEX_POINT('',#179593);
#37939=VERTEX_POINT('',#179595);
#37940=VERTEX_POINT('',#179597);
#37941=VERTEX_POINT('',#179599);
#37942=VERTEX_POINT('',#179603);
#37943=VERTEX_POINT('',#179605);
#37944=VERTEX_POINT('',#179609);
#37945=VERTEX_POINT('',#179610);
#37946=VERTEX_POINT('',#179612);
#37947=VERTEX_POINT('',#179614);
#37948=VERTEX_POINT('',#179618);
#37949=VERTEX_POINT('',#179619);
#37950=VERTEX_POINT('',#179621);
#37951=VERTEX_POINT('',#179623);
#37952=VERTEX_POINT('',#179625);
#37953=VERTEX_POINT('',#179627);
#37954=VERTEX_POINT('',#179631);
#37955=VERTEX_POINT('',#179633);
#37956=VERTEX_POINT('',#179649);
#37957=VERTEX_POINT('',#179650);
#37958=VERTEX_POINT('',#179652);
#37959=VERTEX_POINT('',#179654);
#37960=VERTEX_POINT('',#179656);
#37961=VERTEX_POINT('',#179658);
#37962=VERTEX_POINT('',#179662);
#37963=VERTEX_POINT('',#179664);
#37964=VERTEX_POINT('',#179668);
#37965=VERTEX_POINT('',#179669);
#37966=VERTEX_POINT('',#179671);
#37967=VERTEX_POINT('',#179673);
#37968=VERTEX_POINT('',#179677);
#37969=VERTEX_POINT('',#179678);
#37970=VERTEX_POINT('',#179680);
#37971=VERTEX_POINT('',#179682);
#37972=VERTEX_POINT('',#179684);
#37973=VERTEX_POINT('',#179686);
#37974=VERTEX_POINT('',#179690);
#37975=VERTEX_POINT('',#179692);
#37976=VERTEX_POINT('',#179708);
#37977=VERTEX_POINT('',#179709);
#37978=VERTEX_POINT('',#179711);
#37979=VERTEX_POINT('',#179713);
#37980=VERTEX_POINT('',#179715);
#37981=VERTEX_POINT('',#179717);
#37982=VERTEX_POINT('',#179721);
#37983=VERTEX_POINT('',#179723);
#37984=VERTEX_POINT('',#179727);
#37985=VERTEX_POINT('',#179728);
#37986=VERTEX_POINT('',#179730);
#37987=VERTEX_POINT('',#179732);
#37988=VERTEX_POINT('',#179736);
#37989=VERTEX_POINT('',#179737);
#37990=VERTEX_POINT('',#179739);
#37991=VERTEX_POINT('',#179741);
#37992=VERTEX_POINT('',#179743);
#37993=VERTEX_POINT('',#179745);
#37994=VERTEX_POINT('',#179749);
#37995=VERTEX_POINT('',#179751);
#37996=VERTEX_POINT('',#179767);
#37997=VERTEX_POINT('',#179768);
#37998=VERTEX_POINT('',#179770);
#37999=VERTEX_POINT('',#179772);
#38000=VERTEX_POINT('',#179774);
#38001=VERTEX_POINT('',#179776);
#38002=VERTEX_POINT('',#179780);
#38003=VERTEX_POINT('',#179782);
#38004=VERTEX_POINT('',#179786);
#38005=VERTEX_POINT('',#179787);
#38006=VERTEX_POINT('',#179789);
#38007=VERTEX_POINT('',#179791);
#38008=VERTEX_POINT('',#179795);
#38009=VERTEX_POINT('',#179796);
#38010=VERTEX_POINT('',#179798);
#38011=VERTEX_POINT('',#179800);
#38012=VERTEX_POINT('',#179802);
#38013=VERTEX_POINT('',#179804);
#38014=VERTEX_POINT('',#179808);
#38015=VERTEX_POINT('',#179810);
#38016=VERTEX_POINT('',#179826);
#38017=VERTEX_POINT('',#179827);
#38018=VERTEX_POINT('',#179829);
#38019=VERTEX_POINT('',#179831);
#38020=VERTEX_POINT('',#179833);
#38021=VERTEX_POINT('',#179835);
#38022=VERTEX_POINT('',#179839);
#38023=VERTEX_POINT('',#179841);
#38024=VERTEX_POINT('',#179845);
#38025=VERTEX_POINT('',#179846);
#38026=VERTEX_POINT('',#179848);
#38027=VERTEX_POINT('',#179850);
#38028=VERTEX_POINT('',#179854);
#38029=VERTEX_POINT('',#179855);
#38030=VERTEX_POINT('',#179857);
#38031=VERTEX_POINT('',#179859);
#38032=VERTEX_POINT('',#179861);
#38033=VERTEX_POINT('',#179863);
#38034=VERTEX_POINT('',#179867);
#38035=VERTEX_POINT('',#179869);
#38036=VERTEX_POINT('',#179885);
#38037=VERTEX_POINT('',#179886);
#38038=VERTEX_POINT('',#179888);
#38039=VERTEX_POINT('',#179890);
#38040=VERTEX_POINT('',#179892);
#38041=VERTEX_POINT('',#179894);
#38042=VERTEX_POINT('',#179898);
#38043=VERTEX_POINT('',#179900);
#38044=VERTEX_POINT('',#179904);
#38045=VERTEX_POINT('',#179905);
#38046=VERTEX_POINT('',#179907);
#38047=VERTEX_POINT('',#179909);
#38048=VERTEX_POINT('',#179913);
#38049=VERTEX_POINT('',#179914);
#38050=VERTEX_POINT('',#179916);
#38051=VERTEX_POINT('',#179918);
#38052=VERTEX_POINT('',#179920);
#38053=VERTEX_POINT('',#179922);
#38054=VERTEX_POINT('',#179926);
#38055=VERTEX_POINT('',#179928);
#38056=VERTEX_POINT('',#179944);
#38057=VERTEX_POINT('',#179945);
#38058=VERTEX_POINT('',#179947);
#38059=VERTEX_POINT('',#179949);
#38060=VERTEX_POINT('',#179951);
#38061=VERTEX_POINT('',#179953);
#38062=VERTEX_POINT('',#179957);
#38063=VERTEX_POINT('',#179959);
#38064=VERTEX_POINT('',#179963);
#38065=VERTEX_POINT('',#179964);
#38066=VERTEX_POINT('',#179966);
#38067=VERTEX_POINT('',#179968);
#38068=VERTEX_POINT('',#179972);
#38069=VERTEX_POINT('',#179973);
#38070=VERTEX_POINT('',#179975);
#38071=VERTEX_POINT('',#179977);
#38072=VERTEX_POINT('',#179979);
#38073=VERTEX_POINT('',#179981);
#38074=VERTEX_POINT('',#179985);
#38075=VERTEX_POINT('',#179987);
#38076=VERTEX_POINT('',#180003);
#38077=VERTEX_POINT('',#180004);
#38078=VERTEX_POINT('',#180006);
#38079=VERTEX_POINT('',#180008);
#38080=VERTEX_POINT('',#180010);
#38081=VERTEX_POINT('',#180012);
#38082=VERTEX_POINT('',#180016);
#38083=VERTEX_POINT('',#180018);
#38084=VERTEX_POINT('',#180022);
#38085=VERTEX_POINT('',#180023);
#38086=VERTEX_POINT('',#180025);
#38087=VERTEX_POINT('',#180027);
#38088=VERTEX_POINT('',#180031);
#38089=VERTEX_POINT('',#180032);
#38090=VERTEX_POINT('',#180034);
#38091=VERTEX_POINT('',#180036);
#38092=VERTEX_POINT('',#180038);
#38093=VERTEX_POINT('',#180040);
#38094=VERTEX_POINT('',#180044);
#38095=VERTEX_POINT('',#180046);
#38096=VERTEX_POINT('',#180062);
#38097=VERTEX_POINT('',#180063);
#38098=VERTEX_POINT('',#180065);
#38099=VERTEX_POINT('',#180067);
#38100=VERTEX_POINT('',#180069);
#38101=VERTEX_POINT('',#180071);
#38102=VERTEX_POINT('',#180075);
#38103=VERTEX_POINT('',#180077);
#38104=VERTEX_POINT('',#180081);
#38105=VERTEX_POINT('',#180082);
#38106=VERTEX_POINT('',#180084);
#38107=VERTEX_POINT('',#180086);
#38108=VERTEX_POINT('',#180090);
#38109=VERTEX_POINT('',#180091);
#38110=VERTEX_POINT('',#180093);
#38111=VERTEX_POINT('',#180095);
#38112=VERTEX_POINT('',#180097);
#38113=VERTEX_POINT('',#180099);
#38114=VERTEX_POINT('',#180103);
#38115=VERTEX_POINT('',#180105);
#38116=VERTEX_POINT('',#180121);
#38117=VERTEX_POINT('',#180122);
#38118=VERTEX_POINT('',#180124);
#38119=VERTEX_POINT('',#180126);
#38120=VERTEX_POINT('',#180128);
#38121=VERTEX_POINT('',#180130);
#38122=VERTEX_POINT('',#180134);
#38123=VERTEX_POINT('',#180136);
#38124=VERTEX_POINT('',#180140);
#38125=VERTEX_POINT('',#180141);
#38126=VERTEX_POINT('',#180143);
#38127=VERTEX_POINT('',#180145);
#38128=VERTEX_POINT('',#180149);
#38129=VERTEX_POINT('',#180150);
#38130=VERTEX_POINT('',#180152);
#38131=VERTEX_POINT('',#180154);
#38132=VERTEX_POINT('',#180156);
#38133=VERTEX_POINT('',#180158);
#38134=VERTEX_POINT('',#180162);
#38135=VERTEX_POINT('',#180164);
#38136=VERTEX_POINT('',#180180);
#38137=VERTEX_POINT('',#180181);
#38138=VERTEX_POINT('',#180183);
#38139=VERTEX_POINT('',#180185);
#38140=VERTEX_POINT('',#180187);
#38141=VERTEX_POINT('',#180189);
#38142=VERTEX_POINT('',#180193);
#38143=VERTEX_POINT('',#180195);
#38144=VERTEX_POINT('',#180199);
#38145=VERTEX_POINT('',#180200);
#38146=VERTEX_POINT('',#180202);
#38147=VERTEX_POINT('',#180204);
#38148=VERTEX_POINT('',#180208);
#38149=VERTEX_POINT('',#180209);
#38150=VERTEX_POINT('',#180211);
#38151=VERTEX_POINT('',#180213);
#38152=VERTEX_POINT('',#180215);
#38153=VERTEX_POINT('',#180217);
#38154=VERTEX_POINT('',#180221);
#38155=VERTEX_POINT('',#180223);
#38156=VERTEX_POINT('',#180239);
#38157=VERTEX_POINT('',#180240);
#38158=VERTEX_POINT('',#180242);
#38159=VERTEX_POINT('',#180244);
#38160=VERTEX_POINT('',#180246);
#38161=VERTEX_POINT('',#180248);
#38162=VERTEX_POINT('',#180252);
#38163=VERTEX_POINT('',#180254);
#38164=VERTEX_POINT('',#180258);
#38165=VERTEX_POINT('',#180259);
#38166=VERTEX_POINT('',#180261);
#38167=VERTEX_POINT('',#180263);
#38168=VERTEX_POINT('',#180267);
#38169=VERTEX_POINT('',#180268);
#38170=VERTEX_POINT('',#180270);
#38171=VERTEX_POINT('',#180272);
#38172=VERTEX_POINT('',#180274);
#38173=VERTEX_POINT('',#180276);
#38174=VERTEX_POINT('',#180280);
#38175=VERTEX_POINT('',#180282);
#38176=VERTEX_POINT('',#180298);
#38177=VERTEX_POINT('',#180299);
#38178=VERTEX_POINT('',#180301);
#38179=VERTEX_POINT('',#180303);
#38180=VERTEX_POINT('',#180305);
#38181=VERTEX_POINT('',#180307);
#38182=VERTEX_POINT('',#180311);
#38183=VERTEX_POINT('',#180313);
#38184=VERTEX_POINT('',#180317);
#38185=VERTEX_POINT('',#180318);
#38186=VERTEX_POINT('',#180320);
#38187=VERTEX_POINT('',#180322);
#38188=VERTEX_POINT('',#180326);
#38189=VERTEX_POINT('',#180327);
#38190=VERTEX_POINT('',#180329);
#38191=VERTEX_POINT('',#180331);
#38192=VERTEX_POINT('',#180333);
#38193=VERTEX_POINT('',#180335);
#38194=VERTEX_POINT('',#180339);
#38195=VERTEX_POINT('',#180341);
#38196=VERTEX_POINT('',#180357);
#38197=VERTEX_POINT('',#180358);
#38198=VERTEX_POINT('',#180360);
#38199=VERTEX_POINT('',#180362);
#38200=VERTEX_POINT('',#180364);
#38201=VERTEX_POINT('',#180366);
#38202=VERTEX_POINT('',#180370);
#38203=VERTEX_POINT('',#180372);
#38204=VERTEX_POINT('',#180376);
#38205=VERTEX_POINT('',#180377);
#38206=VERTEX_POINT('',#180379);
#38207=VERTEX_POINT('',#180381);
#38208=VERTEX_POINT('',#180385);
#38209=VERTEX_POINT('',#180386);
#38210=VERTEX_POINT('',#180388);
#38211=VERTEX_POINT('',#180390);
#38212=VERTEX_POINT('',#180392);
#38213=VERTEX_POINT('',#180394);
#38214=VERTEX_POINT('',#180398);
#38215=VERTEX_POINT('',#180400);
#38216=VERTEX_POINT('',#180416);
#38217=VERTEX_POINT('',#180417);
#38218=VERTEX_POINT('',#180419);
#38219=VERTEX_POINT('',#180421);
#38220=VERTEX_POINT('',#180423);
#38221=VERTEX_POINT('',#180425);
#38222=VERTEX_POINT('',#180429);
#38223=VERTEX_POINT('',#180431);
#38224=VERTEX_POINT('',#180435);
#38225=VERTEX_POINT('',#180436);
#38226=VERTEX_POINT('',#180438);
#38227=VERTEX_POINT('',#180440);
#38228=VERTEX_POINT('',#180444);
#38229=VERTEX_POINT('',#180445);
#38230=VERTEX_POINT('',#180447);
#38231=VERTEX_POINT('',#180449);
#38232=VERTEX_POINT('',#180451);
#38233=VERTEX_POINT('',#180453);
#38234=VERTEX_POINT('',#180457);
#38235=VERTEX_POINT('',#180459);
#38236=VERTEX_POINT('',#180475);
#38237=VERTEX_POINT('',#180476);
#38238=VERTEX_POINT('',#180478);
#38239=VERTEX_POINT('',#180480);
#38240=VERTEX_POINT('',#180482);
#38241=VERTEX_POINT('',#180484);
#38242=VERTEX_POINT('',#180488);
#38243=VERTEX_POINT('',#180490);
#38244=VERTEX_POINT('',#180494);
#38245=VERTEX_POINT('',#180495);
#38246=VERTEX_POINT('',#180497);
#38247=VERTEX_POINT('',#180499);
#38248=VERTEX_POINT('',#180503);
#38249=VERTEX_POINT('',#180504);
#38250=VERTEX_POINT('',#180506);
#38251=VERTEX_POINT('',#180508);
#38252=VERTEX_POINT('',#180510);
#38253=VERTEX_POINT('',#180512);
#38254=VERTEX_POINT('',#180516);
#38255=VERTEX_POINT('',#180518);
#38256=VERTEX_POINT('',#180534);
#38257=VERTEX_POINT('',#180535);
#38258=VERTEX_POINT('',#180537);
#38259=VERTEX_POINT('',#180539);
#38260=VERTEX_POINT('',#180541);
#38261=VERTEX_POINT('',#180543);
#38262=VERTEX_POINT('',#180547);
#38263=VERTEX_POINT('',#180549);
#38264=VERTEX_POINT('',#180553);
#38265=VERTEX_POINT('',#180554);
#38266=VERTEX_POINT('',#180556);
#38267=VERTEX_POINT('',#180558);
#38268=VERTEX_POINT('',#180562);
#38269=VERTEX_POINT('',#180563);
#38270=VERTEX_POINT('',#180565);
#38271=VERTEX_POINT('',#180567);
#38272=VERTEX_POINT('',#180569);
#38273=VERTEX_POINT('',#180571);
#38274=VERTEX_POINT('',#180575);
#38275=VERTEX_POINT('',#180577);
#38276=VERTEX_POINT('',#180593);
#38277=VERTEX_POINT('',#180594);
#38278=VERTEX_POINT('',#180596);
#38279=VERTEX_POINT('',#180598);
#38280=VERTEX_POINT('',#180600);
#38281=VERTEX_POINT('',#180602);
#38282=VERTEX_POINT('',#180606);
#38283=VERTEX_POINT('',#180608);
#38284=VERTEX_POINT('',#180612);
#38285=VERTEX_POINT('',#180613);
#38286=VERTEX_POINT('',#180615);
#38287=VERTEX_POINT('',#180617);
#38288=VERTEX_POINT('',#180621);
#38289=VERTEX_POINT('',#180622);
#38290=VERTEX_POINT('',#180624);
#38291=VERTEX_POINT('',#180626);
#38292=VERTEX_POINT('',#180628);
#38293=VERTEX_POINT('',#180630);
#38294=VERTEX_POINT('',#180634);
#38295=VERTEX_POINT('',#180636);
#38296=VERTEX_POINT('',#180652);
#38297=VERTEX_POINT('',#180653);
#38298=VERTEX_POINT('',#180655);
#38299=VERTEX_POINT('',#180657);
#38300=VERTEX_POINT('',#180659);
#38301=VERTEX_POINT('',#180661);
#38302=VERTEX_POINT('',#180665);
#38303=VERTEX_POINT('',#180667);
#38304=VERTEX_POINT('',#180671);
#38305=VERTEX_POINT('',#180672);
#38306=VERTEX_POINT('',#180674);
#38307=VERTEX_POINT('',#180676);
#38308=VERTEX_POINT('',#180680);
#38309=VERTEX_POINT('',#180681);
#38310=VERTEX_POINT('',#180683);
#38311=VERTEX_POINT('',#180685);
#38312=VERTEX_POINT('',#180687);
#38313=VERTEX_POINT('',#180689);
#38314=VERTEX_POINT('',#180693);
#38315=VERTEX_POINT('',#180695);
#38316=VERTEX_POINT('',#180711);
#38317=VERTEX_POINT('',#180712);
#38318=VERTEX_POINT('',#180714);
#38319=VERTEX_POINT('',#180716);
#38320=VERTEX_POINT('',#180718);
#38321=VERTEX_POINT('',#180720);
#38322=VERTEX_POINT('',#180724);
#38323=VERTEX_POINT('',#180726);
#38324=VERTEX_POINT('',#180730);
#38325=VERTEX_POINT('',#180731);
#38326=VERTEX_POINT('',#180733);
#38327=VERTEX_POINT('',#180735);
#38328=VERTEX_POINT('',#180739);
#38329=VERTEX_POINT('',#180740);
#38330=VERTEX_POINT('',#180742);
#38331=VERTEX_POINT('',#180744);
#38332=VERTEX_POINT('',#180746);
#38333=VERTEX_POINT('',#180748);
#38334=VERTEX_POINT('',#180752);
#38335=VERTEX_POINT('',#180754);
#38336=VERTEX_POINT('',#180770);
#38337=VERTEX_POINT('',#180771);
#38338=VERTEX_POINT('',#180773);
#38339=VERTEX_POINT('',#180775);
#38340=VERTEX_POINT('',#180777);
#38341=VERTEX_POINT('',#180779);
#38342=VERTEX_POINT('',#180783);
#38343=VERTEX_POINT('',#180785);
#38344=VERTEX_POINT('',#180789);
#38345=VERTEX_POINT('',#180790);
#38346=VERTEX_POINT('',#180792);
#38347=VERTEX_POINT('',#180794);
#38348=VERTEX_POINT('',#180798);
#38349=VERTEX_POINT('',#180799);
#38350=VERTEX_POINT('',#180801);
#38351=VERTEX_POINT('',#180803);
#38352=VERTEX_POINT('',#180805);
#38353=VERTEX_POINT('',#180807);
#38354=VERTEX_POINT('',#180811);
#38355=VERTEX_POINT('',#180813);
#38356=VERTEX_POINT('',#180829);
#38357=VERTEX_POINT('',#180830);
#38358=VERTEX_POINT('',#180832);
#38359=VERTEX_POINT('',#180834);
#38360=VERTEX_POINT('',#180836);
#38361=VERTEX_POINT('',#180838);
#38362=VERTEX_POINT('',#180842);
#38363=VERTEX_POINT('',#180844);
#38364=VERTEX_POINT('',#180848);
#38365=VERTEX_POINT('',#180849);
#38366=VERTEX_POINT('',#180851);
#38367=VERTEX_POINT('',#180853);
#38368=VERTEX_POINT('',#180857);
#38369=VERTEX_POINT('',#180858);
#38370=VERTEX_POINT('',#180860);
#38371=VERTEX_POINT('',#180862);
#38372=VERTEX_POINT('',#180864);
#38373=VERTEX_POINT('',#180866);
#38374=VERTEX_POINT('',#180870);
#38375=VERTEX_POINT('',#180872);
#38376=VERTEX_POINT('',#180888);
#38377=VERTEX_POINT('',#180889);
#38378=VERTEX_POINT('',#180891);
#38379=VERTEX_POINT('',#180893);
#38380=VERTEX_POINT('',#180895);
#38381=VERTEX_POINT('',#180897);
#38382=VERTEX_POINT('',#180901);
#38383=VERTEX_POINT('',#180903);
#38384=VERTEX_POINT('',#180907);
#38385=VERTEX_POINT('',#180908);
#38386=VERTEX_POINT('',#180910);
#38387=VERTEX_POINT('',#180912);
#38388=VERTEX_POINT('',#180916);
#38389=VERTEX_POINT('',#180917);
#38390=VERTEX_POINT('',#180919);
#38391=VERTEX_POINT('',#180921);
#38392=VERTEX_POINT('',#180923);
#38393=VERTEX_POINT('',#180925);
#38394=VERTEX_POINT('',#180929);
#38395=VERTEX_POINT('',#180931);
#38396=VERTEX_POINT('',#180947);
#38397=VERTEX_POINT('',#180948);
#38398=VERTEX_POINT('',#180950);
#38399=VERTEX_POINT('',#180952);
#38400=VERTEX_POINT('',#180954);
#38401=VERTEX_POINT('',#180956);
#38402=VERTEX_POINT('',#180960);
#38403=VERTEX_POINT('',#180962);
#38404=VERTEX_POINT('',#180966);
#38405=VERTEX_POINT('',#180967);
#38406=VERTEX_POINT('',#180969);
#38407=VERTEX_POINT('',#180971);
#38408=VERTEX_POINT('',#180975);
#38409=VERTEX_POINT('',#180976);
#38410=VERTEX_POINT('',#180978);
#38411=VERTEX_POINT('',#180980);
#38412=VERTEX_POINT('',#180982);
#38413=VERTEX_POINT('',#180984);
#38414=VERTEX_POINT('',#180988);
#38415=VERTEX_POINT('',#180990);
#38416=VERTEX_POINT('',#181006);
#38417=VERTEX_POINT('',#181007);
#38418=VERTEX_POINT('',#181009);
#38419=VERTEX_POINT('',#181011);
#38420=VERTEX_POINT('',#181013);
#38421=VERTEX_POINT('',#181015);
#38422=VERTEX_POINT('',#181019);
#38423=VERTEX_POINT('',#181021);
#38424=VERTEX_POINT('',#181025);
#38425=VERTEX_POINT('',#181026);
#38426=VERTEX_POINT('',#181028);
#38427=VERTEX_POINT('',#181030);
#38428=VERTEX_POINT('',#181034);
#38429=VERTEX_POINT('',#181035);
#38430=VERTEX_POINT('',#181037);
#38431=VERTEX_POINT('',#181039);
#38432=VERTEX_POINT('',#181041);
#38433=VERTEX_POINT('',#181043);
#38434=VERTEX_POINT('',#181047);
#38435=VERTEX_POINT('',#181049);
#38436=VERTEX_POINT('',#181065);
#38437=VERTEX_POINT('',#181066);
#38438=VERTEX_POINT('',#181068);
#38439=VERTEX_POINT('',#181070);
#38440=VERTEX_POINT('',#181072);
#38441=VERTEX_POINT('',#181074);
#38442=VERTEX_POINT('',#181078);
#38443=VERTEX_POINT('',#181080);
#38444=VERTEX_POINT('',#181084);
#38445=VERTEX_POINT('',#181085);
#38446=VERTEX_POINT('',#181087);
#38447=VERTEX_POINT('',#181089);
#38448=VERTEX_POINT('',#181093);
#38449=VERTEX_POINT('',#181094);
#38450=VERTEX_POINT('',#181096);
#38451=VERTEX_POINT('',#181098);
#38452=VERTEX_POINT('',#181100);
#38453=VERTEX_POINT('',#181102);
#38454=VERTEX_POINT('',#181106);
#38455=VERTEX_POINT('',#181108);
#38456=VERTEX_POINT('',#181124);
#38457=VERTEX_POINT('',#181125);
#38458=VERTEX_POINT('',#181127);
#38459=VERTEX_POINT('',#181129);
#38460=VERTEX_POINT('',#181131);
#38461=VERTEX_POINT('',#181133);
#38462=VERTEX_POINT('',#181137);
#38463=VERTEX_POINT('',#181139);
#38464=VERTEX_POINT('',#181143);
#38465=VERTEX_POINT('',#181144);
#38466=VERTEX_POINT('',#181146);
#38467=VERTEX_POINT('',#181148);
#38468=VERTEX_POINT('',#181152);
#38469=VERTEX_POINT('',#181153);
#38470=VERTEX_POINT('',#181155);
#38471=VERTEX_POINT('',#181157);
#38472=VERTEX_POINT('',#181159);
#38473=VERTEX_POINT('',#181161);
#38474=VERTEX_POINT('',#181165);
#38475=VERTEX_POINT('',#181167);
#38476=VERTEX_POINT('',#181183);
#38477=VERTEX_POINT('',#181184);
#38478=VERTEX_POINT('',#181186);
#38479=VERTEX_POINT('',#181188);
#38480=VERTEX_POINT('',#181190);
#38481=VERTEX_POINT('',#181192);
#38482=VERTEX_POINT('',#181196);
#38483=VERTEX_POINT('',#181198);
#38484=VERTEX_POINT('',#181202);
#38485=VERTEX_POINT('',#181203);
#38486=VERTEX_POINT('',#181205);
#38487=VERTEX_POINT('',#181207);
#38488=VERTEX_POINT('',#181211);
#38489=VERTEX_POINT('',#181212);
#38490=VERTEX_POINT('',#181214);
#38491=VERTEX_POINT('',#181216);
#38492=VERTEX_POINT('',#181218);
#38493=VERTEX_POINT('',#181220);
#38494=VERTEX_POINT('',#181224);
#38495=VERTEX_POINT('',#181226);
#38496=VERTEX_POINT('',#181242);
#38497=VERTEX_POINT('',#181243);
#38498=VERTEX_POINT('',#181245);
#38499=VERTEX_POINT('',#181247);
#38500=VERTEX_POINT('',#181249);
#38501=VERTEX_POINT('',#181251);
#38502=VERTEX_POINT('',#181255);
#38503=VERTEX_POINT('',#181257);
#38504=VERTEX_POINT('',#181261);
#38505=VERTEX_POINT('',#181262);
#38506=VERTEX_POINT('',#181264);
#38507=VERTEX_POINT('',#181266);
#38508=VERTEX_POINT('',#181270);
#38509=VERTEX_POINT('',#181271);
#38510=VERTEX_POINT('',#181273);
#38511=VERTEX_POINT('',#181275);
#38512=VERTEX_POINT('',#181277);
#38513=VERTEX_POINT('',#181279);
#38514=VERTEX_POINT('',#181283);
#38515=VERTEX_POINT('',#181285);
#38516=VERTEX_POINT('',#181301);
#38517=VERTEX_POINT('',#181302);
#38518=VERTEX_POINT('',#181304);
#38519=VERTEX_POINT('',#181306);
#38520=VERTEX_POINT('',#181308);
#38521=VERTEX_POINT('',#181310);
#38522=VERTEX_POINT('',#181314);
#38523=VERTEX_POINT('',#181316);
#38524=VERTEX_POINT('',#181320);
#38525=VERTEX_POINT('',#181321);
#38526=VERTEX_POINT('',#181323);
#38527=VERTEX_POINT('',#181325);
#38528=VERTEX_POINT('',#181329);
#38529=VERTEX_POINT('',#181330);
#38530=VERTEX_POINT('',#181332);
#38531=VERTEX_POINT('',#181334);
#38532=VERTEX_POINT('',#181336);
#38533=VERTEX_POINT('',#181338);
#38534=VERTEX_POINT('',#181342);
#38535=VERTEX_POINT('',#181344);
#38536=VERTEX_POINT('',#181360);
#38537=VERTEX_POINT('',#181361);
#38538=VERTEX_POINT('',#181363);
#38539=VERTEX_POINT('',#181365);
#38540=VERTEX_POINT('',#181367);
#38541=VERTEX_POINT('',#181369);
#38542=VERTEX_POINT('',#181373);
#38543=VERTEX_POINT('',#181375);
#38544=VERTEX_POINT('',#181379);
#38545=VERTEX_POINT('',#181380);
#38546=VERTEX_POINT('',#181382);
#38547=VERTEX_POINT('',#181384);
#38548=VERTEX_POINT('',#181388);
#38549=VERTEX_POINT('',#181389);
#38550=VERTEX_POINT('',#181391);
#38551=VERTEX_POINT('',#181393);
#38552=VERTEX_POINT('',#181395);
#38553=VERTEX_POINT('',#181397);
#38554=VERTEX_POINT('',#181401);
#38555=VERTEX_POINT('',#181403);
#38556=VERTEX_POINT('',#181419);
#38557=VERTEX_POINT('',#181420);
#38558=VERTEX_POINT('',#181422);
#38559=VERTEX_POINT('',#181424);
#38560=VERTEX_POINT('',#181426);
#38561=VERTEX_POINT('',#181428);
#38562=VERTEX_POINT('',#181432);
#38563=VERTEX_POINT('',#181434);
#38564=VERTEX_POINT('',#181438);
#38565=VERTEX_POINT('',#181439);
#38566=VERTEX_POINT('',#181441);
#38567=VERTEX_POINT('',#181443);
#38568=VERTEX_POINT('',#181447);
#38569=VERTEX_POINT('',#181448);
#38570=VERTEX_POINT('',#181450);
#38571=VERTEX_POINT('',#181452);
#38572=VERTEX_POINT('',#181454);
#38573=VERTEX_POINT('',#181456);
#38574=VERTEX_POINT('',#181460);
#38575=VERTEX_POINT('',#181462);
#38576=VERTEX_POINT('',#181478);
#38577=VERTEX_POINT('',#181479);
#38578=VERTEX_POINT('',#181481);
#38579=VERTEX_POINT('',#181483);
#38580=VERTEX_POINT('',#181485);
#38581=VERTEX_POINT('',#181487);
#38582=VERTEX_POINT('',#181491);
#38583=VERTEX_POINT('',#181493);
#38584=VERTEX_POINT('',#181497);
#38585=VERTEX_POINT('',#181498);
#38586=VERTEX_POINT('',#181500);
#38587=VERTEX_POINT('',#181502);
#38588=VERTEX_POINT('',#181506);
#38589=VERTEX_POINT('',#181507);
#38590=VERTEX_POINT('',#181509);
#38591=VERTEX_POINT('',#181511);
#38592=VERTEX_POINT('',#181513);
#38593=VERTEX_POINT('',#181515);
#38594=VERTEX_POINT('',#181519);
#38595=VERTEX_POINT('',#181521);
#38596=VERTEX_POINT('',#181537);
#38597=VERTEX_POINT('',#181538);
#38598=VERTEX_POINT('',#181540);
#38599=VERTEX_POINT('',#181542);
#38600=VERTEX_POINT('',#181544);
#38601=VERTEX_POINT('',#181546);
#38602=VERTEX_POINT('',#181550);
#38603=VERTEX_POINT('',#181552);
#38604=VERTEX_POINT('',#181556);
#38605=VERTEX_POINT('',#181557);
#38606=VERTEX_POINT('',#181559);
#38607=VERTEX_POINT('',#181561);
#38608=VERTEX_POINT('',#181565);
#38609=VERTEX_POINT('',#181566);
#38610=VERTEX_POINT('',#181568);
#38611=VERTEX_POINT('',#181570);
#38612=VERTEX_POINT('',#181572);
#38613=VERTEX_POINT('',#181574);
#38614=VERTEX_POINT('',#181578);
#38615=VERTEX_POINT('',#181580);
#38616=VERTEX_POINT('',#181596);
#38617=VERTEX_POINT('',#181597);
#38618=VERTEX_POINT('',#181599);
#38619=VERTEX_POINT('',#181601);
#38620=VERTEX_POINT('',#181603);
#38621=VERTEX_POINT('',#181605);
#38622=VERTEX_POINT('',#181609);
#38623=VERTEX_POINT('',#181611);
#38624=VERTEX_POINT('',#181615);
#38625=VERTEX_POINT('',#181616);
#38626=VERTEX_POINT('',#181618);
#38627=VERTEX_POINT('',#181620);
#38628=VERTEX_POINT('',#181624);
#38629=VERTEX_POINT('',#181625);
#38630=VERTEX_POINT('',#181627);
#38631=VERTEX_POINT('',#181629);
#38632=VERTEX_POINT('',#181631);
#38633=VERTEX_POINT('',#181633);
#38634=VERTEX_POINT('',#181637);
#38635=VERTEX_POINT('',#181639);
#38636=VERTEX_POINT('',#181655);
#38637=VERTEX_POINT('',#181656);
#38638=VERTEX_POINT('',#181658);
#38639=VERTEX_POINT('',#181660);
#38640=VERTEX_POINT('',#181662);
#38641=VERTEX_POINT('',#181664);
#38642=VERTEX_POINT('',#181668);
#38643=VERTEX_POINT('',#181670);
#38644=VERTEX_POINT('',#181674);
#38645=VERTEX_POINT('',#181675);
#38646=VERTEX_POINT('',#181677);
#38647=VERTEX_POINT('',#181679);
#38648=VERTEX_POINT('',#181683);
#38649=VERTEX_POINT('',#181684);
#38650=VERTEX_POINT('',#181686);
#38651=VERTEX_POINT('',#181688);
#38652=VERTEX_POINT('',#181690);
#38653=VERTEX_POINT('',#181692);
#38654=VERTEX_POINT('',#181696);
#38655=VERTEX_POINT('',#181698);
#38656=VERTEX_POINT('',#181714);
#38657=VERTEX_POINT('',#181715);
#38658=VERTEX_POINT('',#181717);
#38659=VERTEX_POINT('',#181719);
#38660=VERTEX_POINT('',#181721);
#38661=VERTEX_POINT('',#181723);
#38662=VERTEX_POINT('',#181727);
#38663=VERTEX_POINT('',#181729);
#38664=VERTEX_POINT('',#181733);
#38665=VERTEX_POINT('',#181734);
#38666=VERTEX_POINT('',#181736);
#38667=VERTEX_POINT('',#181738);
#38668=VERTEX_POINT('',#181742);
#38669=VERTEX_POINT('',#181743);
#38670=VERTEX_POINT('',#181745);
#38671=VERTEX_POINT('',#181747);
#38672=VERTEX_POINT('',#181749);
#38673=VERTEX_POINT('',#181751);
#38674=VERTEX_POINT('',#181755);
#38675=VERTEX_POINT('',#181757);
#38676=VERTEX_POINT('',#181773);
#38677=VERTEX_POINT('',#181774);
#38678=VERTEX_POINT('',#181776);
#38679=VERTEX_POINT('',#181778);
#38680=VERTEX_POINT('',#181780);
#38681=VERTEX_POINT('',#181782);
#38682=VERTEX_POINT('',#181786);
#38683=VERTEX_POINT('',#181788);
#38684=VERTEX_POINT('',#181792);
#38685=VERTEX_POINT('',#181793);
#38686=VERTEX_POINT('',#181795);
#38687=VERTEX_POINT('',#181797);
#38688=VERTEX_POINT('',#181801);
#38689=VERTEX_POINT('',#181802);
#38690=VERTEX_POINT('',#181804);
#38691=VERTEX_POINT('',#181806);
#38692=VERTEX_POINT('',#181808);
#38693=VERTEX_POINT('',#181810);
#38694=VERTEX_POINT('',#181814);
#38695=VERTEX_POINT('',#181816);
#38696=VERTEX_POINT('',#181832);
#38697=VERTEX_POINT('',#181833);
#38698=VERTEX_POINT('',#181835);
#38699=VERTEX_POINT('',#181837);
#38700=VERTEX_POINT('',#181839);
#38701=VERTEX_POINT('',#181841);
#38702=VERTEX_POINT('',#181845);
#38703=VERTEX_POINT('',#181847);
#38704=VERTEX_POINT('',#181851);
#38705=VERTEX_POINT('',#181852);
#38706=VERTEX_POINT('',#181854);
#38707=VERTEX_POINT('',#181856);
#38708=VERTEX_POINT('',#181860);
#38709=VERTEX_POINT('',#181861);
#38710=VERTEX_POINT('',#181863);
#38711=VERTEX_POINT('',#181865);
#38712=VERTEX_POINT('',#181867);
#38713=VERTEX_POINT('',#181869);
#38714=VERTEX_POINT('',#181873);
#38715=VERTEX_POINT('',#181875);
#38716=VERTEX_POINT('',#181891);
#38717=VERTEX_POINT('',#181892);
#38718=VERTEX_POINT('',#181894);
#38719=VERTEX_POINT('',#181896);
#38720=VERTEX_POINT('',#181898);
#38721=VERTEX_POINT('',#181900);
#38722=VERTEX_POINT('',#181904);
#38723=VERTEX_POINT('',#181906);
#38724=VERTEX_POINT('',#181910);
#38725=VERTEX_POINT('',#181911);
#38726=VERTEX_POINT('',#181913);
#38727=VERTEX_POINT('',#181915);
#38728=VERTEX_POINT('',#181919);
#38729=VERTEX_POINT('',#181920);
#38730=VERTEX_POINT('',#181922);
#38731=VERTEX_POINT('',#181924);
#38732=VERTEX_POINT('',#181926);
#38733=VERTEX_POINT('',#181928);
#38734=VERTEX_POINT('',#181932);
#38735=VERTEX_POINT('',#181934);
#38736=VERTEX_POINT('',#181951);
#38737=VERTEX_POINT('',#181952);
#38738=VERTEX_POINT('',#181954);
#38739=VERTEX_POINT('',#181956);
#38740=VERTEX_POINT('',#181958);
#38741=VERTEX_POINT('',#181960);
#38742=VERTEX_POINT('',#181964);
#38743=VERTEX_POINT('',#181966);
#38744=VERTEX_POINT('',#181970);
#38745=VERTEX_POINT('',#181971);
#38746=VERTEX_POINT('',#181973);
#38747=VERTEX_POINT('',#181975);
#38748=VERTEX_POINT('',#181979);
#38749=VERTEX_POINT('',#181980);
#38750=VERTEX_POINT('',#181982);
#38751=VERTEX_POINT('',#181984);
#38752=VERTEX_POINT('',#181986);
#38753=VERTEX_POINT('',#181988);
#38754=VERTEX_POINT('',#181992);
#38755=VERTEX_POINT('',#181994);
#38756=VERTEX_POINT('',#182012);
#38757=VERTEX_POINT('',#182013);
#38758=VERTEX_POINT('',#182015);
#38759=VERTEX_POINT('',#182017);
#38760=VERTEX_POINT('',#182021);
#38761=VERTEX_POINT('',#182022);
#38762=VERTEX_POINT('',#182024);
#38763=VERTEX_POINT('',#182026);
#38764=VERTEX_POINT('',#182028);
#38765=VERTEX_POINT('',#182030);
#38766=VERTEX_POINT('',#182032);
#38767=VERTEX_POINT('',#182034);
#38768=VERTEX_POINT('',#182036);
#38769=VERTEX_POINT('',#182038);
#38770=VERTEX_POINT('',#182040);
#38771=VERTEX_POINT('',#182042);
#38772=VERTEX_POINT('',#182046);
#38773=VERTEX_POINT('',#182047);
#38774=VERTEX_POINT('',#182049);
#38775=VERTEX_POINT('',#182051);
#38776=VERTEX_POINT('',#182053);
#38777=VERTEX_POINT('',#182055);
#38778=VERTEX_POINT('',#182057);
#38779=VERTEX_POINT('',#182059);
#38780=VERTEX_POINT('',#182061);
#38781=VERTEX_POINT('',#182063);
#38782=VERTEX_POINT('',#182065);
#38783=VERTEX_POINT('',#182067);
#38784=VERTEX_POINT('',#182487);
#38785=VERTEX_POINT('',#182488);
#38786=VERTEX_POINT('',#182490);
#38787=VERTEX_POINT('',#182492);
#38788=VERTEX_POINT('',#182496);
#38789=VERTEX_POINT('',#182497);
#38790=VERTEX_POINT('',#182499);
#38791=VERTEX_POINT('',#182501);
#38792=VERTEX_POINT('',#182503);
#38793=VERTEX_POINT('',#182505);
#38794=VERTEX_POINT('',#182507);
#38795=VERTEX_POINT('',#182509);
#38796=VERTEX_POINT('',#182511);
#38797=VERTEX_POINT('',#182513);
#38798=VERTEX_POINT('',#182515);
#38799=VERTEX_POINT('',#182517);
#38800=VERTEX_POINT('',#182521);
#38801=VERTEX_POINT('',#182522);
#38802=VERTEX_POINT('',#182524);
#38803=VERTEX_POINT('',#182526);
#38804=VERTEX_POINT('',#182528);
#38805=VERTEX_POINT('',#182530);
#38806=VERTEX_POINT('',#182532);
#38807=VERTEX_POINT('',#182534);
#38808=VERTEX_POINT('',#182536);
#38809=VERTEX_POINT('',#182538);
#38810=VERTEX_POINT('',#182540);
#38811=VERTEX_POINT('',#182542);
#38812=VERTEX_POINT('',#182546);
#38813=VERTEX_POINT('',#182547);
#38814=VERTEX_POINT('',#182549);
#38815=VERTEX_POINT('',#182551);
#38816=VERTEX_POINT('',#182555);
#38817=VERTEX_POINT('',#182556);
#38818=VERTEX_POINT('',#182558);
#38819=VERTEX_POINT('',#182560);
#38820=VERTEX_POINT('',#182562);
#38821=VERTEX_POINT('',#182564);
#38822=VERTEX_POINT('',#182566);
#38823=VERTEX_POINT('',#182568);
#38824=VERTEX_POINT('',#182570);
#38825=VERTEX_POINT('',#182572);
#38826=VERTEX_POINT('',#182574);
#38827=VERTEX_POINT('',#182576);
#38828=VERTEX_POINT('',#182580);
#38829=VERTEX_POINT('',#182581);
#38830=VERTEX_POINT('',#182583);
#38831=VERTEX_POINT('',#182585);
#38832=VERTEX_POINT('',#182587);
#38833=VERTEX_POINT('',#182589);
#38834=VERTEX_POINT('',#182591);
#38835=VERTEX_POINT('',#182593);
#38836=VERTEX_POINT('',#182595);
#38837=VERTEX_POINT('',#182597);
#38838=VERTEX_POINT('',#182599);
#38839=VERTEX_POINT('',#182601);
#38840=VERTEX_POINT('',#182605);
#38841=VERTEX_POINT('',#182606);
#38842=VERTEX_POINT('',#182608);
#38843=VERTEX_POINT('',#182610);
#38844=VERTEX_POINT('',#182614);
#38845=VERTEX_POINT('',#182615);
#38846=VERTEX_POINT('',#182617);
#38847=VERTEX_POINT('',#182619);
#38848=VERTEX_POINT('',#182621);
#38849=VERTEX_POINT('',#182623);
#38850=VERTEX_POINT('',#182625);
#38851=VERTEX_POINT('',#182627);
#38852=VERTEX_POINT('',#182629);
#38853=VERTEX_POINT('',#182631);
#38854=VERTEX_POINT('',#182633);
#38855=VERTEX_POINT('',#182635);
#38856=VERTEX_POINT('',#182639);
#38857=VERTEX_POINT('',#182640);
#38858=VERTEX_POINT('',#182642);
#38859=VERTEX_POINT('',#182644);
#38860=VERTEX_POINT('',#182646);
#38861=VERTEX_POINT('',#182648);
#38862=VERTEX_POINT('',#182650);
#38863=VERTEX_POINT('',#182652);
#38864=VERTEX_POINT('',#182654);
#38865=VERTEX_POINT('',#182656);
#38866=VERTEX_POINT('',#182658);
#38867=VERTEX_POINT('',#182660);
#38868=VERTEX_POINT('',#182664);
#38869=VERTEX_POINT('',#182665);
#38870=VERTEX_POINT('',#182667);
#38871=VERTEX_POINT('',#182669);
#38872=VERTEX_POINT('',#182673);
#38873=VERTEX_POINT('',#182674);
#38874=VERTEX_POINT('',#182676);
#38875=VERTEX_POINT('',#182678);
#38876=VERTEX_POINT('',#182680);
#38877=VERTEX_POINT('',#182682);
#38878=VERTEX_POINT('',#182684);
#38879=VERTEX_POINT('',#182686);
#38880=VERTEX_POINT('',#182688);
#38881=VERTEX_POINT('',#182690);
#38882=VERTEX_POINT('',#182692);
#38883=VERTEX_POINT('',#182694);
#38884=VERTEX_POINT('',#182698);
#38885=VERTEX_POINT('',#182699);
#38886=VERTEX_POINT('',#182701);
#38887=VERTEX_POINT('',#182703);
#38888=VERTEX_POINT('',#182705);
#38889=VERTEX_POINT('',#182707);
#38890=VERTEX_POINT('',#182709);
#38891=VERTEX_POINT('',#182711);
#38892=VERTEX_POINT('',#182713);
#38893=VERTEX_POINT('',#182715);
#38894=VERTEX_POINT('',#182717);
#38895=VERTEX_POINT('',#182719);
#38896=VERTEX_POINT('',#182723);
#38897=VERTEX_POINT('',#182724);
#38898=VERTEX_POINT('',#182726);
#38899=VERTEX_POINT('',#182728);
#38900=VERTEX_POINT('',#182732);
#38901=VERTEX_POINT('',#182733);
#38902=VERTEX_POINT('',#182735);
#38903=VERTEX_POINT('',#182737);
#38904=VERTEX_POINT('',#182739);
#38905=VERTEX_POINT('',#182741);
#38906=VERTEX_POINT('',#182743);
#38907=VERTEX_POINT('',#182745);
#38908=VERTEX_POINT('',#182747);
#38909=VERTEX_POINT('',#182749);
#38910=VERTEX_POINT('',#182751);
#38911=VERTEX_POINT('',#182753);
#38912=VERTEX_POINT('',#182757);
#38913=VERTEX_POINT('',#182758);
#38914=VERTEX_POINT('',#182760);
#38915=VERTEX_POINT('',#182762);
#38916=VERTEX_POINT('',#182764);
#38917=VERTEX_POINT('',#182766);
#38918=VERTEX_POINT('',#182768);
#38919=VERTEX_POINT('',#182770);
#38920=VERTEX_POINT('',#182772);
#38921=VERTEX_POINT('',#182774);
#38922=VERTEX_POINT('',#182776);
#38923=VERTEX_POINT('',#182778);
#38924=VERTEX_POINT('',#182782);
#38925=VERTEX_POINT('',#182783);
#38926=VERTEX_POINT('',#182785);
#38927=VERTEX_POINT('',#182787);
#38928=VERTEX_POINT('',#182791);
#38929=VERTEX_POINT('',#182792);
#38930=VERTEX_POINT('',#182794);
#38931=VERTEX_POINT('',#182796);
#38932=VERTEX_POINT('',#182798);
#38933=VERTEX_POINT('',#182800);
#38934=VERTEX_POINT('',#182802);
#38935=VERTEX_POINT('',#182804);
#38936=VERTEX_POINT('',#182806);
#38937=VERTEX_POINT('',#182808);
#38938=VERTEX_POINT('',#182810);
#38939=VERTEX_POINT('',#182812);
#38940=VERTEX_POINT('',#182816);
#38941=VERTEX_POINT('',#182817);
#38942=VERTEX_POINT('',#182819);
#38943=VERTEX_POINT('',#182821);
#38944=VERTEX_POINT('',#182823);
#38945=VERTEX_POINT('',#182825);
#38946=VERTEX_POINT('',#182827);
#38947=VERTEX_POINT('',#182829);
#38948=VERTEX_POINT('',#182831);
#38949=VERTEX_POINT('',#182833);
#38950=VERTEX_POINT('',#182835);
#38951=VERTEX_POINT('',#182837);
#38952=VERTEX_POINT('',#182841);
#38953=VERTEX_POINT('',#182842);
#38954=VERTEX_POINT('',#182844);
#38955=VERTEX_POINT('',#182846);
#38956=VERTEX_POINT('',#182850);
#38957=VERTEX_POINT('',#182851);
#38958=VERTEX_POINT('',#182853);
#38959=VERTEX_POINT('',#182855);
#38960=VERTEX_POINT('',#182857);
#38961=VERTEX_POINT('',#182859);
#38962=VERTEX_POINT('',#182861);
#38963=VERTEX_POINT('',#182863);
#38964=VERTEX_POINT('',#182865);
#38965=VERTEX_POINT('',#182867);
#38966=VERTEX_POINT('',#182869);
#38967=VERTEX_POINT('',#182871);
#38968=VERTEX_POINT('',#182875);
#38969=VERTEX_POINT('',#182876);
#38970=VERTEX_POINT('',#182878);
#38971=VERTEX_POINT('',#182880);
#38972=VERTEX_POINT('',#182882);
#38973=VERTEX_POINT('',#182884);
#38974=VERTEX_POINT('',#182886);
#38975=VERTEX_POINT('',#182888);
#38976=VERTEX_POINT('',#182890);
#38977=VERTEX_POINT('',#182892);
#38978=VERTEX_POINT('',#182894);
#38979=VERTEX_POINT('',#182896);
#38980=VERTEX_POINT('',#182900);
#38981=VERTEX_POINT('',#182901);
#38982=VERTEX_POINT('',#182903);
#38983=VERTEX_POINT('',#182905);
#38984=VERTEX_POINT('',#182909);
#38985=VERTEX_POINT('',#182910);
#38986=VERTEX_POINT('',#182912);
#38987=VERTEX_POINT('',#182914);
#38988=VERTEX_POINT('',#182916);
#38989=VERTEX_POINT('',#182918);
#38990=VERTEX_POINT('',#182920);
#38991=VERTEX_POINT('',#182922);
#38992=VERTEX_POINT('',#182924);
#38993=VERTEX_POINT('',#182926);
#38994=VERTEX_POINT('',#182928);
#38995=VERTEX_POINT('',#182930);
#38996=VERTEX_POINT('',#182934);
#38997=VERTEX_POINT('',#182935);
#38998=VERTEX_POINT('',#182937);
#38999=VERTEX_POINT('',#182939);
#39000=VERTEX_POINT('',#182941);
#39001=VERTEX_POINT('',#182943);
#39002=VERTEX_POINT('',#182945);
#39003=VERTEX_POINT('',#182947);
#39004=VERTEX_POINT('',#182949);
#39005=VERTEX_POINT('',#182951);
#39006=VERTEX_POINT('',#182953);
#39007=VERTEX_POINT('',#182955);
#39008=VERTEX_POINT('',#182959);
#39009=VERTEX_POINT('',#182960);
#39010=VERTEX_POINT('',#182962);
#39011=VERTEX_POINT('',#182964);
#39012=VERTEX_POINT('',#182968);
#39013=VERTEX_POINT('',#182969);
#39014=VERTEX_POINT('',#182971);
#39015=VERTEX_POINT('',#182973);
#39016=VERTEX_POINT('',#182975);
#39017=VERTEX_POINT('',#182977);
#39018=VERTEX_POINT('',#182979);
#39019=VERTEX_POINT('',#182981);
#39020=VERTEX_POINT('',#182983);
#39021=VERTEX_POINT('',#182985);
#39022=VERTEX_POINT('',#182987);
#39023=VERTEX_POINT('',#182989);
#39024=VERTEX_POINT('',#182993);
#39025=VERTEX_POINT('',#182994);
#39026=VERTEX_POINT('',#182996);
#39027=VERTEX_POINT('',#182998);
#39028=VERTEX_POINT('',#183000);
#39029=VERTEX_POINT('',#183002);
#39030=VERTEX_POINT('',#183004);
#39031=VERTEX_POINT('',#183006);
#39032=VERTEX_POINT('',#183008);
#39033=VERTEX_POINT('',#183010);
#39034=VERTEX_POINT('',#183012);
#39035=VERTEX_POINT('',#183014);
#39036=VERTEX_POINT('',#183018);
#39037=VERTEX_POINT('',#183019);
#39038=VERTEX_POINT('',#183021);
#39039=VERTEX_POINT('',#183023);
#39040=VERTEX_POINT('',#183027);
#39041=VERTEX_POINT('',#183028);
#39042=VERTEX_POINT('',#183030);
#39043=VERTEX_POINT('',#183032);
#39044=VERTEX_POINT('',#183034);
#39045=VERTEX_POINT('',#183036);
#39046=VERTEX_POINT('',#183038);
#39047=VERTEX_POINT('',#183040);
#39048=VERTEX_POINT('',#183042);
#39049=VERTEX_POINT('',#183044);
#39050=VERTEX_POINT('',#183046);
#39051=VERTEX_POINT('',#183048);
#39052=VERTEX_POINT('',#183052);
#39053=VERTEX_POINT('',#183053);
#39054=VERTEX_POINT('',#183055);
#39055=VERTEX_POINT('',#183057);
#39056=VERTEX_POINT('',#183059);
#39057=VERTEX_POINT('',#183061);
#39058=VERTEX_POINT('',#183063);
#39059=VERTEX_POINT('',#183065);
#39060=VERTEX_POINT('',#183067);
#39061=VERTEX_POINT('',#183069);
#39062=VERTEX_POINT('',#183071);
#39063=VERTEX_POINT('',#183073);
#39064=VERTEX_POINT('',#183077);
#39065=VERTEX_POINT('',#183078);
#39066=VERTEX_POINT('',#183080);
#39067=VERTEX_POINT('',#183082);
#39068=VERTEX_POINT('',#183086);
#39069=VERTEX_POINT('',#183087);
#39070=VERTEX_POINT('',#183089);
#39071=VERTEX_POINT('',#183091);
#39072=VERTEX_POINT('',#183093);
#39073=VERTEX_POINT('',#183095);
#39074=VERTEX_POINT('',#183097);
#39075=VERTEX_POINT('',#183099);
#39076=VERTEX_POINT('',#183101);
#39077=VERTEX_POINT('',#183103);
#39078=VERTEX_POINT('',#183105);
#39079=VERTEX_POINT('',#183107);
#39080=VERTEX_POINT('',#183111);
#39081=VERTEX_POINT('',#183112);
#39082=VERTEX_POINT('',#183114);
#39083=VERTEX_POINT('',#183116);
#39084=VERTEX_POINT('',#183118);
#39085=VERTEX_POINT('',#183120);
#39086=VERTEX_POINT('',#183122);
#39087=VERTEX_POINT('',#183124);
#39088=VERTEX_POINT('',#183126);
#39089=VERTEX_POINT('',#183128);
#39090=VERTEX_POINT('',#183130);
#39091=VERTEX_POINT('',#183132);
#39092=VERTEX_POINT('',#183136);
#39093=VERTEX_POINT('',#183137);
#39094=VERTEX_POINT('',#183139);
#39095=VERTEX_POINT('',#183141);
#39096=VERTEX_POINT('',#183145);
#39097=VERTEX_POINT('',#183146);
#39098=VERTEX_POINT('',#183148);
#39099=VERTEX_POINT('',#183150);
#39100=VERTEX_POINT('',#183152);
#39101=VERTEX_POINT('',#183154);
#39102=VERTEX_POINT('',#183156);
#39103=VERTEX_POINT('',#183158);
#39104=VERTEX_POINT('',#183160);
#39105=VERTEX_POINT('',#183162);
#39106=VERTEX_POINT('',#183164);
#39107=VERTEX_POINT('',#183166);
#39108=VERTEX_POINT('',#183170);
#39109=VERTEX_POINT('',#183171);
#39110=VERTEX_POINT('',#183173);
#39111=VERTEX_POINT('',#183175);
#39112=VERTEX_POINT('',#183177);
#39113=VERTEX_POINT('',#183179);
#39114=VERTEX_POINT('',#183181);
#39115=VERTEX_POINT('',#183183);
#39116=VERTEX_POINT('',#183185);
#39117=VERTEX_POINT('',#183187);
#39118=VERTEX_POINT('',#183189);
#39119=VERTEX_POINT('',#183191);
#39120=VERTEX_POINT('',#183195);
#39121=VERTEX_POINT('',#183196);
#39122=VERTEX_POINT('',#183198);
#39123=VERTEX_POINT('',#183200);
#39124=VERTEX_POINT('',#183204);
#39125=VERTEX_POINT('',#183205);
#39126=VERTEX_POINT('',#183207);
#39127=VERTEX_POINT('',#183209);
#39128=VERTEX_POINT('',#183211);
#39129=VERTEX_POINT('',#183213);
#39130=VERTEX_POINT('',#183215);
#39131=VERTEX_POINT('',#183217);
#39132=VERTEX_POINT('',#183219);
#39133=VERTEX_POINT('',#183221);
#39134=VERTEX_POINT('',#183223);
#39135=VERTEX_POINT('',#183225);
#39136=VERTEX_POINT('',#183229);
#39137=VERTEX_POINT('',#183230);
#39138=VERTEX_POINT('',#183232);
#39139=VERTEX_POINT('',#183234);
#39140=VERTEX_POINT('',#183236);
#39141=VERTEX_POINT('',#183238);
#39142=VERTEX_POINT('',#183240);
#39143=VERTEX_POINT('',#183242);
#39144=VERTEX_POINT('',#183244);
#39145=VERTEX_POINT('',#183246);
#39146=VERTEX_POINT('',#183248);
#39147=VERTEX_POINT('',#183250);
#39148=VERTEX_POINT('',#183254);
#39149=VERTEX_POINT('',#183255);
#39150=VERTEX_POINT('',#183257);
#39151=VERTEX_POINT('',#183259);
#39152=VERTEX_POINT('',#183263);
#39153=VERTEX_POINT('',#183264);
#39154=VERTEX_POINT('',#183266);
#39155=VERTEX_POINT('',#183268);
#39156=VERTEX_POINT('',#183270);
#39157=VERTEX_POINT('',#183272);
#39158=VERTEX_POINT('',#183274);
#39159=VERTEX_POINT('',#183276);
#39160=VERTEX_POINT('',#183278);
#39161=VERTEX_POINT('',#183280);
#39162=VERTEX_POINT('',#183282);
#39163=VERTEX_POINT('',#183284);
#39164=VERTEX_POINT('',#183288);
#39165=VERTEX_POINT('',#183289);
#39166=VERTEX_POINT('',#183291);
#39167=VERTEX_POINT('',#183293);
#39168=VERTEX_POINT('',#183295);
#39169=VERTEX_POINT('',#183297);
#39170=VERTEX_POINT('',#183299);
#39171=VERTEX_POINT('',#183301);
#39172=VERTEX_POINT('',#183303);
#39173=VERTEX_POINT('',#183305);
#39174=VERTEX_POINT('',#183307);
#39175=VERTEX_POINT('',#183309);
#39176=VERTEX_POINT('',#183313);
#39177=VERTEX_POINT('',#183314);
#39178=VERTEX_POINT('',#183316);
#39179=VERTEX_POINT('',#183318);
#39180=VERTEX_POINT('',#183322);
#39181=VERTEX_POINT('',#183323);
#39182=VERTEX_POINT('',#183325);
#39183=VERTEX_POINT('',#183327);
#39184=VERTEX_POINT('',#183329);
#39185=VERTEX_POINT('',#183331);
#39186=VERTEX_POINT('',#183333);
#39187=VERTEX_POINT('',#183335);
#39188=VERTEX_POINT('',#183337);
#39189=VERTEX_POINT('',#183339);
#39190=VERTEX_POINT('',#183341);
#39191=VERTEX_POINT('',#183343);
#39192=VERTEX_POINT('',#183347);
#39193=VERTEX_POINT('',#183348);
#39194=VERTEX_POINT('',#183350);
#39195=VERTEX_POINT('',#183352);
#39196=VERTEX_POINT('',#183354);
#39197=VERTEX_POINT('',#183356);
#39198=VERTEX_POINT('',#183358);
#39199=VERTEX_POINT('',#183360);
#39200=VERTEX_POINT('',#183362);
#39201=VERTEX_POINT('',#183364);
#39202=VERTEX_POINT('',#183366);
#39203=VERTEX_POINT('',#183368);
#39204=VERTEX_POINT('',#183372);
#39205=VERTEX_POINT('',#183373);
#39206=VERTEX_POINT('',#183375);
#39207=VERTEX_POINT('',#183377);
#39208=VERTEX_POINT('',#183381);
#39209=VERTEX_POINT('',#183382);
#39210=VERTEX_POINT('',#183384);
#39211=VERTEX_POINT('',#183386);
#39212=VERTEX_POINT('',#183388);
#39213=VERTEX_POINT('',#183390);
#39214=VERTEX_POINT('',#183392);
#39215=VERTEX_POINT('',#183394);
#39216=VERTEX_POINT('',#183396);
#39217=VERTEX_POINT('',#183398);
#39218=VERTEX_POINT('',#183400);
#39219=VERTEX_POINT('',#183402);
#39220=VERTEX_POINT('',#183406);
#39221=VERTEX_POINT('',#183407);
#39222=VERTEX_POINT('',#183409);
#39223=VERTEX_POINT('',#183411);
#39224=VERTEX_POINT('',#183413);
#39225=VERTEX_POINT('',#183415);
#39226=VERTEX_POINT('',#183417);
#39227=VERTEX_POINT('',#183419);
#39228=VERTEX_POINT('',#183421);
#39229=VERTEX_POINT('',#183423);
#39230=VERTEX_POINT('',#183425);
#39231=VERTEX_POINT('',#183427);
#39232=VERTEX_POINT('',#183431);
#39233=VERTEX_POINT('',#183432);
#39234=VERTEX_POINT('',#183434);
#39235=VERTEX_POINT('',#183436);
#39236=VERTEX_POINT('',#183440);
#39237=VERTEX_POINT('',#183441);
#39238=VERTEX_POINT('',#183443);
#39239=VERTEX_POINT('',#183445);
#39240=VERTEX_POINT('',#183447);
#39241=VERTEX_POINT('',#183449);
#39242=VERTEX_POINT('',#183451);
#39243=VERTEX_POINT('',#183453);
#39244=VERTEX_POINT('',#183455);
#39245=VERTEX_POINT('',#183457);
#39246=VERTEX_POINT('',#183459);
#39247=VERTEX_POINT('',#183461);
#39248=VERTEX_POINT('',#183465);
#39249=VERTEX_POINT('',#183466);
#39250=VERTEX_POINT('',#183468);
#39251=VERTEX_POINT('',#183470);
#39252=VERTEX_POINT('',#183472);
#39253=VERTEX_POINT('',#183474);
#39254=VERTEX_POINT('',#183476);
#39255=VERTEX_POINT('',#183478);
#39256=VERTEX_POINT('',#183480);
#39257=VERTEX_POINT('',#183482);
#39258=VERTEX_POINT('',#183484);
#39259=VERTEX_POINT('',#183486);
#39260=VERTEX_POINT('',#183490);
#39261=VERTEX_POINT('',#183491);
#39262=VERTEX_POINT('',#183493);
#39263=VERTEX_POINT('',#183495);
#39264=VERTEX_POINT('',#183499);
#39265=VERTEX_POINT('',#183500);
#39266=VERTEX_POINT('',#183502);
#39267=VERTEX_POINT('',#183504);
#39268=VERTEX_POINT('',#183506);
#39269=VERTEX_POINT('',#183508);
#39270=VERTEX_POINT('',#183510);
#39271=VERTEX_POINT('',#183512);
#39272=VERTEX_POINT('',#183514);
#39273=VERTEX_POINT('',#183516);
#39274=VERTEX_POINT('',#183518);
#39275=VERTEX_POINT('',#183520);
#39276=VERTEX_POINT('',#183524);
#39277=VERTEX_POINT('',#183525);
#39278=VERTEX_POINT('',#183527);
#39279=VERTEX_POINT('',#183529);
#39280=VERTEX_POINT('',#183531);
#39281=VERTEX_POINT('',#183533);
#39282=VERTEX_POINT('',#183535);
#39283=VERTEX_POINT('',#183537);
#39284=VERTEX_POINT('',#183539);
#39285=VERTEX_POINT('',#183541);
#39286=VERTEX_POINT('',#183543);
#39287=VERTEX_POINT('',#183545);
#39288=VERTEX_POINT('',#183549);
#39289=VERTEX_POINT('',#183550);
#39290=VERTEX_POINT('',#183552);
#39291=VERTEX_POINT('',#183554);
#39292=VERTEX_POINT('',#183558);
#39293=VERTEX_POINT('',#183559);
#39294=VERTEX_POINT('',#183561);
#39295=VERTEX_POINT('',#183563);
#39296=VERTEX_POINT('',#183565);
#39297=VERTEX_POINT('',#183567);
#39298=VERTEX_POINT('',#183569);
#39299=VERTEX_POINT('',#183571);
#39300=VERTEX_POINT('',#183573);
#39301=VERTEX_POINT('',#183575);
#39302=VERTEX_POINT('',#183577);
#39303=VERTEX_POINT('',#183579);
#39304=VERTEX_POINT('',#183583);
#39305=VERTEX_POINT('',#183584);
#39306=VERTEX_POINT('',#183586);
#39307=VERTEX_POINT('',#183588);
#39308=VERTEX_POINT('',#183590);
#39309=VERTEX_POINT('',#183592);
#39310=VERTEX_POINT('',#183594);
#39311=VERTEX_POINT('',#183596);
#39312=VERTEX_POINT('',#183598);
#39313=VERTEX_POINT('',#183600);
#39314=VERTEX_POINT('',#183602);
#39315=VERTEX_POINT('',#183604);
#39316=VERTEX_POINT('',#183608);
#39317=VERTEX_POINT('',#183609);
#39318=VERTEX_POINT('',#183611);
#39319=VERTEX_POINT('',#183613);
#39320=VERTEX_POINT('',#183617);
#39321=VERTEX_POINT('',#183618);
#39322=VERTEX_POINT('',#183620);
#39323=VERTEX_POINT('',#183622);
#39324=VERTEX_POINT('',#183624);
#39325=VERTEX_POINT('',#183626);
#39326=VERTEX_POINT('',#183628);
#39327=VERTEX_POINT('',#183630);
#39328=VERTEX_POINT('',#183632);
#39329=VERTEX_POINT('',#183634);
#39330=VERTEX_POINT('',#183636);
#39331=VERTEX_POINT('',#183638);
#39332=VERTEX_POINT('',#183642);
#39333=VERTEX_POINT('',#183643);
#39334=VERTEX_POINT('',#183645);
#39335=VERTEX_POINT('',#183647);
#39336=VERTEX_POINT('',#183649);
#39337=VERTEX_POINT('',#183651);
#39338=VERTEX_POINT('',#183653);
#39339=VERTEX_POINT('',#183655);
#39340=VERTEX_POINT('',#183657);
#39341=VERTEX_POINT('',#183659);
#39342=VERTEX_POINT('',#183661);
#39343=VERTEX_POINT('',#183663);
#39344=VERTEX_POINT('',#183667);
#39345=VERTEX_POINT('',#183668);
#39346=VERTEX_POINT('',#183670);
#39347=VERTEX_POINT('',#183672);
#39348=VERTEX_POINT('',#183676);
#39349=VERTEX_POINT('',#183677);
#39350=VERTEX_POINT('',#183679);
#39351=VERTEX_POINT('',#183681);
#39352=VERTEX_POINT('',#183683);
#39353=VERTEX_POINT('',#183685);
#39354=VERTEX_POINT('',#183687);
#39355=VERTEX_POINT('',#183689);
#39356=VERTEX_POINT('',#183691);
#39357=VERTEX_POINT('',#183693);
#39358=VERTEX_POINT('',#183695);
#39359=VERTEX_POINT('',#183697);
#39360=VERTEX_POINT('',#183701);
#39361=VERTEX_POINT('',#183702);
#39362=VERTEX_POINT('',#183704);
#39363=VERTEX_POINT('',#183706);
#39364=VERTEX_POINT('',#183708);
#39365=VERTEX_POINT('',#183710);
#39366=VERTEX_POINT('',#183712);
#39367=VERTEX_POINT('',#183714);
#39368=VERTEX_POINT('',#183716);
#39369=VERTEX_POINT('',#183718);
#39370=VERTEX_POINT('',#183720);
#39371=VERTEX_POINT('',#183722);
#39372=VERTEX_POINT('',#183726);
#39373=VERTEX_POINT('',#183727);
#39374=VERTEX_POINT('',#183729);
#39375=VERTEX_POINT('',#183731);
#39376=VERTEX_POINT('',#183735);
#39377=VERTEX_POINT('',#183736);
#39378=VERTEX_POINT('',#183738);
#39379=VERTEX_POINT('',#183740);
#39380=VERTEX_POINT('',#183742);
#39381=VERTEX_POINT('',#183744);
#39382=VERTEX_POINT('',#183746);
#39383=VERTEX_POINT('',#183748);
#39384=VERTEX_POINT('',#183750);
#39385=VERTEX_POINT('',#183752);
#39386=VERTEX_POINT('',#183754);
#39387=VERTEX_POINT('',#183756);
#39388=VERTEX_POINT('',#183760);
#39389=VERTEX_POINT('',#183761);
#39390=VERTEX_POINT('',#183763);
#39391=VERTEX_POINT('',#183765);
#39392=VERTEX_POINT('',#183767);
#39393=VERTEX_POINT('',#183769);
#39394=VERTEX_POINT('',#183771);
#39395=VERTEX_POINT('',#183773);
#39396=VERTEX_POINT('',#183775);
#39397=VERTEX_POINT('',#183777);
#39398=VERTEX_POINT('',#183779);
#39399=VERTEX_POINT('',#183781);
#39400=VERTEX_POINT('',#183785);
#39401=VERTEX_POINT('',#183786);
#39402=VERTEX_POINT('',#183788);
#39403=VERTEX_POINT('',#183790);
#39404=VERTEX_POINT('',#183794);
#39405=VERTEX_POINT('',#183795);
#39406=VERTEX_POINT('',#183797);
#39407=VERTEX_POINT('',#183799);
#39408=VERTEX_POINT('',#183801);
#39409=VERTEX_POINT('',#183803);
#39410=VERTEX_POINT('',#183805);
#39411=VERTEX_POINT('',#183807);
#39412=VERTEX_POINT('',#183809);
#39413=VERTEX_POINT('',#183811);
#39414=VERTEX_POINT('',#183813);
#39415=VERTEX_POINT('',#183815);
#39416=VERTEX_POINT('',#183819);
#39417=VERTEX_POINT('',#183820);
#39418=VERTEX_POINT('',#183822);
#39419=VERTEX_POINT('',#183824);
#39420=VERTEX_POINT('',#183826);
#39421=VERTEX_POINT('',#183828);
#39422=VERTEX_POINT('',#183830);
#39423=VERTEX_POINT('',#183832);
#39424=VERTEX_POINT('',#183834);
#39425=VERTEX_POINT('',#183836);
#39426=VERTEX_POINT('',#183838);
#39427=VERTEX_POINT('',#183840);
#39428=VERTEX_POINT('',#183844);
#39429=VERTEX_POINT('',#183845);
#39430=VERTEX_POINT('',#183847);
#39431=VERTEX_POINT('',#183849);
#39432=VERTEX_POINT('',#183853);
#39433=VERTEX_POINT('',#183854);
#39434=VERTEX_POINT('',#183856);
#39435=VERTEX_POINT('',#183858);
#39436=VERTEX_POINT('',#183860);
#39437=VERTEX_POINT('',#183862);
#39438=VERTEX_POINT('',#183864);
#39439=VERTEX_POINT('',#183866);
#39440=VERTEX_POINT('',#183868);
#39441=VERTEX_POINT('',#183870);
#39442=VERTEX_POINT('',#183872);
#39443=VERTEX_POINT('',#183874);
#39444=VERTEX_POINT('',#183878);
#39445=VERTEX_POINT('',#183879);
#39446=VERTEX_POINT('',#183881);
#39447=VERTEX_POINT('',#183883);
#39448=VERTEX_POINT('',#183885);
#39449=VERTEX_POINT('',#183887);
#39450=VERTEX_POINT('',#183889);
#39451=VERTEX_POINT('',#183891);
#39452=VERTEX_POINT('',#183893);
#39453=VERTEX_POINT('',#183895);
#39454=VERTEX_POINT('',#183897);
#39455=VERTEX_POINT('',#183899);
#39456=VERTEX_POINT('',#183903);
#39457=VERTEX_POINT('',#183904);
#39458=VERTEX_POINT('',#183906);
#39459=VERTEX_POINT('',#183908);
#39460=VERTEX_POINT('',#183912);
#39461=VERTEX_POINT('',#183913);
#39462=VERTEX_POINT('',#183915);
#39463=VERTEX_POINT('',#183917);
#39464=VERTEX_POINT('',#183919);
#39465=VERTEX_POINT('',#183921);
#39466=VERTEX_POINT('',#183923);
#39467=VERTEX_POINT('',#183925);
#39468=VERTEX_POINT('',#183927);
#39469=VERTEX_POINT('',#183929);
#39470=VERTEX_POINT('',#183931);
#39471=VERTEX_POINT('',#183933);
#39472=VERTEX_POINT('',#183937);
#39473=VERTEX_POINT('',#183938);
#39474=VERTEX_POINT('',#183940);
#39475=VERTEX_POINT('',#183942);
#39476=VERTEX_POINT('',#183944);
#39477=VERTEX_POINT('',#183946);
#39478=VERTEX_POINT('',#183948);
#39479=VERTEX_POINT('',#183950);
#39480=VERTEX_POINT('',#183952);
#39481=VERTEX_POINT('',#183954);
#39482=VERTEX_POINT('',#183956);
#39483=VERTEX_POINT('',#183958);
#39484=VERTEX_POINT('',#183962);
#39485=VERTEX_POINT('',#183963);
#39486=VERTEX_POINT('',#183965);
#39487=VERTEX_POINT('',#183967);
#39488=VERTEX_POINT('',#183971);
#39489=VERTEX_POINT('',#183972);
#39490=VERTEX_POINT('',#183974);
#39491=VERTEX_POINT('',#183976);
#39492=VERTEX_POINT('',#183978);
#39493=VERTEX_POINT('',#183980);
#39494=VERTEX_POINT('',#183982);
#39495=VERTEX_POINT('',#183984);
#39496=VERTEX_POINT('',#183986);
#39497=VERTEX_POINT('',#183988);
#39498=VERTEX_POINT('',#183990);
#39499=VERTEX_POINT('',#183992);
#39500=VERTEX_POINT('',#183996);
#39501=VERTEX_POINT('',#183997);
#39502=VERTEX_POINT('',#183999);
#39503=VERTEX_POINT('',#184001);
#39504=VERTEX_POINT('',#184003);
#39505=VERTEX_POINT('',#184005);
#39506=VERTEX_POINT('',#184007);
#39507=VERTEX_POINT('',#184009);
#39508=VERTEX_POINT('',#184011);
#39509=VERTEX_POINT('',#184013);
#39510=VERTEX_POINT('',#184015);
#39511=VERTEX_POINT('',#184017);
#39512=VERTEX_POINT('',#184021);
#39513=VERTEX_POINT('',#184022);
#39514=VERTEX_POINT('',#184024);
#39515=VERTEX_POINT('',#184026);
#39516=VERTEX_POINT('',#184030);
#39517=VERTEX_POINT('',#184031);
#39518=VERTEX_POINT('',#184033);
#39519=VERTEX_POINT('',#184035);
#39520=VERTEX_POINT('',#184037);
#39521=VERTEX_POINT('',#184039);
#39522=VERTEX_POINT('',#184041);
#39523=VERTEX_POINT('',#184043);
#39524=VERTEX_POINT('',#184045);
#39525=VERTEX_POINT('',#184047);
#39526=VERTEX_POINT('',#184049);
#39527=VERTEX_POINT('',#184051);
#39528=VERTEX_POINT('',#184055);
#39529=VERTEX_POINT('',#184056);
#39530=VERTEX_POINT('',#184058);
#39531=VERTEX_POINT('',#184060);
#39532=VERTEX_POINT('',#184062);
#39533=VERTEX_POINT('',#184064);
#39534=VERTEX_POINT('',#184066);
#39535=VERTEX_POINT('',#184068);
#39536=VERTEX_POINT('',#184070);
#39537=VERTEX_POINT('',#184072);
#39538=VERTEX_POINT('',#184074);
#39539=VERTEX_POINT('',#184076);
#39540=VERTEX_POINT('',#184080);
#39541=VERTEX_POINT('',#184081);
#39542=VERTEX_POINT('',#184083);
#39543=VERTEX_POINT('',#184085);
#39544=VERTEX_POINT('',#184089);
#39545=VERTEX_POINT('',#184090);
#39546=VERTEX_POINT('',#184092);
#39547=VERTEX_POINT('',#184094);
#39548=VERTEX_POINT('',#184096);
#39549=VERTEX_POINT('',#184098);
#39550=VERTEX_POINT('',#184100);
#39551=VERTEX_POINT('',#184102);
#39552=VERTEX_POINT('',#184104);
#39553=VERTEX_POINT('',#184106);
#39554=VERTEX_POINT('',#184108);
#39555=VERTEX_POINT('',#184110);
#39556=VERTEX_POINT('',#184114);
#39557=VERTEX_POINT('',#184115);
#39558=VERTEX_POINT('',#184117);
#39559=VERTEX_POINT('',#184119);
#39560=VERTEX_POINT('',#184121);
#39561=VERTEX_POINT('',#184123);
#39562=VERTEX_POINT('',#184125);
#39563=VERTEX_POINT('',#184127);
#39564=VERTEX_POINT('',#184129);
#39565=VERTEX_POINT('',#184131);
#39566=VERTEX_POINT('',#184133);
#39567=VERTEX_POINT('',#184135);
#39568=VERTEX_POINT('',#184139);
#39569=VERTEX_POINT('',#184140);
#39570=VERTEX_POINT('',#184142);
#39571=VERTEX_POINT('',#184144);
#39572=VERTEX_POINT('',#184148);
#39573=VERTEX_POINT('',#184149);
#39574=VERTEX_POINT('',#184151);
#39575=VERTEX_POINT('',#184153);
#39576=VERTEX_POINT('',#184155);
#39577=VERTEX_POINT('',#184157);
#39578=VERTEX_POINT('',#184159);
#39579=VERTEX_POINT('',#184161);
#39580=VERTEX_POINT('',#184163);
#39581=VERTEX_POINT('',#184165);
#39582=VERTEX_POINT('',#184167);
#39583=VERTEX_POINT('',#184169);
#39584=VERTEX_POINT('',#184173);
#39585=VERTEX_POINT('',#184174);
#39586=VERTEX_POINT('',#184176);
#39587=VERTEX_POINT('',#184178);
#39588=VERTEX_POINT('',#184180);
#39589=VERTEX_POINT('',#184182);
#39590=VERTEX_POINT('',#184184);
#39591=VERTEX_POINT('',#184186);
#39592=VERTEX_POINT('',#184188);
#39593=VERTEX_POINT('',#184190);
#39594=VERTEX_POINT('',#184192);
#39595=VERTEX_POINT('',#184194);
#39596=VERTEX_POINT('',#184201);
#39597=VERTEX_POINT('',#184202);
#39598=VERTEX_POINT('',#184204);
#39599=VERTEX_POINT('',#184206);
#39600=VERTEX_POINT('',#184208);
#39601=VERTEX_POINT('',#184210);
#39602=VERTEX_POINT('',#184212);
#39603=VERTEX_POINT('',#184214);
#39604=VERTEX_POINT('',#184216);
#39605=VERTEX_POINT('',#184218);
#39606=VERTEX_POINT('',#184220);
#39607=VERTEX_POINT('',#184222);
#39608=VERTEX_POINT('',#184226);
#39609=VERTEX_POINT('',#184227);
#39610=VERTEX_POINT('',#184229);
#39611=VERTEX_POINT('',#184231);
#39612=VERTEX_POINT('',#184233);
#39613=VERTEX_POINT('',#184235);
#39614=VERTEX_POINT('',#184237);
#39615=VERTEX_POINT('',#184239);
#39616=VERTEX_POINT('',#184241);
#39617=VERTEX_POINT('',#184243);
#39618=VERTEX_POINT('',#184245);
#39619=VERTEX_POINT('',#184247);
#39620=VERTEX_POINT('',#184251);
#39621=VERTEX_POINT('',#184252);
#39622=VERTEX_POINT('',#184254);
#39623=VERTEX_POINT('',#184256);
#39624=VERTEX_POINT('',#184260);
#39625=VERTEX_POINT('',#184261);
#39626=VERTEX_POINT('',#184263);
#39627=VERTEX_POINT('',#184265);
#39628=VERTEX_POINT('',#184267);
#39629=VERTEX_POINT('',#184269);
#39630=VERTEX_POINT('',#184271);
#39631=VERTEX_POINT('',#184273);
#39632=VERTEX_POINT('',#184275);
#39633=VERTEX_POINT('',#184277);
#39634=VERTEX_POINT('',#184279);
#39635=VERTEX_POINT('',#184281);
#39636=VERTEX_POINT('',#184285);
#39637=VERTEX_POINT('',#184286);
#39638=VERTEX_POINT('',#184288);
#39639=VERTEX_POINT('',#184290);
#39640=VERTEX_POINT('',#184292);
#39641=VERTEX_POINT('',#184294);
#39642=VERTEX_POINT('',#184296);
#39643=VERTEX_POINT('',#184298);
#39644=VERTEX_POINT('',#184300);
#39645=VERTEX_POINT('',#184302);
#39646=VERTEX_POINT('',#184304);
#39647=VERTEX_POINT('',#184306);
#39648=VERTEX_POINT('',#184310);
#39649=VERTEX_POINT('',#184311);
#39650=VERTEX_POINT('',#184313);
#39651=VERTEX_POINT('',#184315);
#39652=VERTEX_POINT('',#184319);
#39653=VERTEX_POINT('',#184320);
#39654=VERTEX_POINT('',#184322);
#39655=VERTEX_POINT('',#184324);
#39656=VERTEX_POINT('',#184326);
#39657=VERTEX_POINT('',#184328);
#39658=VERTEX_POINT('',#184330);
#39659=VERTEX_POINT('',#184332);
#39660=VERTEX_POINT('',#184334);
#39661=VERTEX_POINT('',#184336);
#39662=VERTEX_POINT('',#184338);
#39663=VERTEX_POINT('',#184340);
#39664=VERTEX_POINT('',#184344);
#39665=VERTEX_POINT('',#184345);
#39666=VERTEX_POINT('',#184347);
#39667=VERTEX_POINT('',#184349);
#39668=VERTEX_POINT('',#184351);
#39669=VERTEX_POINT('',#184353);
#39670=VERTEX_POINT('',#184355);
#39671=VERTEX_POINT('',#184357);
#39672=VERTEX_POINT('',#184359);
#39673=VERTEX_POINT('',#184361);
#39674=VERTEX_POINT('',#184363);
#39675=VERTEX_POINT('',#184365);
#39676=VERTEX_POINT('',#184369);
#39677=VERTEX_POINT('',#184370);
#39678=VERTEX_POINT('',#184372);
#39679=VERTEX_POINT('',#184374);
#39680=VERTEX_POINT('',#184378);
#39681=VERTEX_POINT('',#184379);
#39682=VERTEX_POINT('',#184381);
#39683=VERTEX_POINT('',#184383);
#39684=VERTEX_POINT('',#184385);
#39685=VERTEX_POINT('',#184387);
#39686=VERTEX_POINT('',#184389);
#39687=VERTEX_POINT('',#184391);
#39688=VERTEX_POINT('',#184393);
#39689=VERTEX_POINT('',#184395);
#39690=VERTEX_POINT('',#184397);
#39691=VERTEX_POINT('',#184399);
#39692=VERTEX_POINT('',#184403);
#39693=VERTEX_POINT('',#184404);
#39694=VERTEX_POINT('',#184406);
#39695=VERTEX_POINT('',#184408);
#39696=VERTEX_POINT('',#184410);
#39697=VERTEX_POINT('',#184412);
#39698=VERTEX_POINT('',#184414);
#39699=VERTEX_POINT('',#184416);
#39700=VERTEX_POINT('',#184418);
#39701=VERTEX_POINT('',#184420);
#39702=VERTEX_POINT('',#184422);
#39703=VERTEX_POINT('',#184424);
#39704=VERTEX_POINT('',#184428);
#39705=VERTEX_POINT('',#184429);
#39706=VERTEX_POINT('',#184431);
#39707=VERTEX_POINT('',#184433);
#39708=VERTEX_POINT('',#184437);
#39709=VERTEX_POINT('',#184438);
#39710=VERTEX_POINT('',#184440);
#39711=VERTEX_POINT('',#184442);
#39712=VERTEX_POINT('',#184444);
#39713=VERTEX_POINT('',#184446);
#39714=VERTEX_POINT('',#184448);
#39715=VERTEX_POINT('',#184450);
#39716=VERTEX_POINT('',#184452);
#39717=VERTEX_POINT('',#184454);
#39718=VERTEX_POINT('',#184456);
#39719=VERTEX_POINT('',#184458);
#39720=VERTEX_POINT('',#184462);
#39721=VERTEX_POINT('',#184463);
#39722=VERTEX_POINT('',#184465);
#39723=VERTEX_POINT('',#184467);
#39724=VERTEX_POINT('',#184469);
#39725=VERTEX_POINT('',#184471);
#39726=VERTEX_POINT('',#184473);
#39727=VERTEX_POINT('',#184475);
#39728=VERTEX_POINT('',#184477);
#39729=VERTEX_POINT('',#184479);
#39730=VERTEX_POINT('',#184481);
#39731=VERTEX_POINT('',#184483);
#39732=VERTEX_POINT('',#184487);
#39733=VERTEX_POINT('',#184488);
#39734=VERTEX_POINT('',#184490);
#39735=VERTEX_POINT('',#184492);
#39736=VERTEX_POINT('',#184496);
#39737=VERTEX_POINT('',#184497);
#39738=VERTEX_POINT('',#184499);
#39739=VERTEX_POINT('',#184501);
#39740=VERTEX_POINT('',#184503);
#39741=VERTEX_POINT('',#184505);
#39742=VERTEX_POINT('',#184507);
#39743=VERTEX_POINT('',#184509);
#39744=VERTEX_POINT('',#184511);
#39745=VERTEX_POINT('',#184513);
#39746=VERTEX_POINT('',#184515);
#39747=VERTEX_POINT('',#184517);
#39748=VERTEX_POINT('',#184521);
#39749=VERTEX_POINT('',#184522);
#39750=VERTEX_POINT('',#184524);
#39751=VERTEX_POINT('',#184526);
#39752=VERTEX_POINT('',#184528);
#39753=VERTEX_POINT('',#184530);
#39754=VERTEX_POINT('',#184532);
#39755=VERTEX_POINT('',#184534);
#39756=VERTEX_POINT('',#184536);
#39757=VERTEX_POINT('',#184538);
#39758=VERTEX_POINT('',#184540);
#39759=VERTEX_POINT('',#184542);
#39760=VERTEX_POINT('',#184546);
#39761=VERTEX_POINT('',#184547);
#39762=VERTEX_POINT('',#184549);
#39763=VERTEX_POINT('',#184551);
#39764=VERTEX_POINT('',#184555);
#39765=VERTEX_POINT('',#184556);
#39766=VERTEX_POINT('',#184558);
#39767=VERTEX_POINT('',#184560);
#39768=VERTEX_POINT('',#184562);
#39769=VERTEX_POINT('',#184564);
#39770=VERTEX_POINT('',#184566);
#39771=VERTEX_POINT('',#184568);
#39772=VERTEX_POINT('',#184570);
#39773=VERTEX_POINT('',#184572);
#39774=VERTEX_POINT('',#184574);
#39775=VERTEX_POINT('',#184576);
#39776=VERTEX_POINT('',#184580);
#39777=VERTEX_POINT('',#184581);
#39778=VERTEX_POINT('',#184583);
#39779=VERTEX_POINT('',#184585);
#39780=VERTEX_POINT('',#184587);
#39781=VERTEX_POINT('',#184589);
#39782=VERTEX_POINT('',#184591);
#39783=VERTEX_POINT('',#184593);
#39784=VERTEX_POINT('',#184595);
#39785=VERTEX_POINT('',#184597);
#39786=VERTEX_POINT('',#184599);
#39787=VERTEX_POINT('',#184601);
#39788=VERTEX_POINT('',#184605);
#39789=VERTEX_POINT('',#184606);
#39790=VERTEX_POINT('',#184608);
#39791=VERTEX_POINT('',#184610);
#39792=VERTEX_POINT('',#184614);
#39793=VERTEX_POINT('',#184615);
#39794=VERTEX_POINT('',#184617);
#39795=VERTEX_POINT('',#184619);
#39796=VERTEX_POINT('',#184621);
#39797=VERTEX_POINT('',#184623);
#39798=VERTEX_POINT('',#184625);
#39799=VERTEX_POINT('',#184627);
#39800=VERTEX_POINT('',#184629);
#39801=VERTEX_POINT('',#184631);
#39802=VERTEX_POINT('',#184633);
#39803=VERTEX_POINT('',#184635);
#39804=VERTEX_POINT('',#184639);
#39805=VERTEX_POINT('',#184640);
#39806=VERTEX_POINT('',#184642);
#39807=VERTEX_POINT('',#184644);
#39808=VERTEX_POINT('',#184646);
#39809=VERTEX_POINT('',#184648);
#39810=VERTEX_POINT('',#184650);
#39811=VERTEX_POINT('',#184652);
#39812=VERTEX_POINT('',#184654);
#39813=VERTEX_POINT('',#184656);
#39814=VERTEX_POINT('',#184658);
#39815=VERTEX_POINT('',#184660);
#39816=VERTEX_POINT('',#184664);
#39817=VERTEX_POINT('',#184665);
#39818=VERTEX_POINT('',#184667);
#39819=VERTEX_POINT('',#184669);
#39820=VERTEX_POINT('',#184673);
#39821=VERTEX_POINT('',#184674);
#39822=VERTEX_POINT('',#184676);
#39823=VERTEX_POINT('',#184678);
#39824=VERTEX_POINT('',#184680);
#39825=VERTEX_POINT('',#184682);
#39826=VERTEX_POINT('',#184684);
#39827=VERTEX_POINT('',#184686);
#39828=VERTEX_POINT('',#184688);
#39829=VERTEX_POINT('',#184690);
#39830=VERTEX_POINT('',#184692);
#39831=VERTEX_POINT('',#184694);
#39832=VERTEX_POINT('',#184698);
#39833=VERTEX_POINT('',#184699);
#39834=VERTEX_POINT('',#184701);
#39835=VERTEX_POINT('',#184703);
#39836=VERTEX_POINT('',#184705);
#39837=VERTEX_POINT('',#184707);
#39838=VERTEX_POINT('',#184709);
#39839=VERTEX_POINT('',#184711);
#39840=VERTEX_POINT('',#184713);
#39841=VERTEX_POINT('',#184715);
#39842=VERTEX_POINT('',#184717);
#39843=VERTEX_POINT('',#184719);
#39844=VERTEX_POINT('',#184723);
#39845=VERTEX_POINT('',#184724);
#39846=VERTEX_POINT('',#184726);
#39847=VERTEX_POINT('',#184728);
#39848=VERTEX_POINT('',#184732);
#39849=VERTEX_POINT('',#184733);
#39850=VERTEX_POINT('',#184735);
#39851=VERTEX_POINT('',#184737);
#39852=VERTEX_POINT('',#184739);
#39853=VERTEX_POINT('',#184741);
#39854=VERTEX_POINT('',#184743);
#39855=VERTEX_POINT('',#184745);
#39856=VERTEX_POINT('',#184747);
#39857=VERTEX_POINT('',#184749);
#39858=VERTEX_POINT('',#184751);
#39859=VERTEX_POINT('',#184753);
#39860=VERTEX_POINT('',#184757);
#39861=VERTEX_POINT('',#184758);
#39862=VERTEX_POINT('',#184760);
#39863=VERTEX_POINT('',#184762);
#39864=VERTEX_POINT('',#184764);
#39865=VERTEX_POINT('',#184766);
#39866=VERTEX_POINT('',#184768);
#39867=VERTEX_POINT('',#184770);
#39868=VERTEX_POINT('',#184772);
#39869=VERTEX_POINT('',#184774);
#39870=VERTEX_POINT('',#184776);
#39871=VERTEX_POINT('',#184778);
#39872=VERTEX_POINT('',#184782);
#39873=VERTEX_POINT('',#184783);
#39874=VERTEX_POINT('',#184785);
#39875=VERTEX_POINT('',#184787);
#39876=VERTEX_POINT('',#184791);
#39877=VERTEX_POINT('',#184792);
#39878=VERTEX_POINT('',#184794);
#39879=VERTEX_POINT('',#184796);
#39880=VERTEX_POINT('',#184798);
#39881=VERTEX_POINT('',#184800);
#39882=VERTEX_POINT('',#184802);
#39883=VERTEX_POINT('',#184804);
#39884=VERTEX_POINT('',#184806);
#39885=VERTEX_POINT('',#184808);
#39886=VERTEX_POINT('',#184810);
#39887=VERTEX_POINT('',#184812);
#39888=VERTEX_POINT('',#184816);
#39889=VERTEX_POINT('',#184817);
#39890=VERTEX_POINT('',#184819);
#39891=VERTEX_POINT('',#184821);
#39892=VERTEX_POINT('',#184823);
#39893=VERTEX_POINT('',#184825);
#39894=VERTEX_POINT('',#184827);
#39895=VERTEX_POINT('',#184829);
#39896=VERTEX_POINT('',#184831);
#39897=VERTEX_POINT('',#184833);
#39898=VERTEX_POINT('',#184835);
#39899=VERTEX_POINT('',#184837);
#39900=VERTEX_POINT('',#184841);
#39901=VERTEX_POINT('',#184842);
#39902=VERTEX_POINT('',#184844);
#39903=VERTEX_POINT('',#184846);
#39904=VERTEX_POINT('',#184850);
#39905=VERTEX_POINT('',#184851);
#39906=VERTEX_POINT('',#184853);
#39907=VERTEX_POINT('',#184855);
#39908=VERTEX_POINT('',#184857);
#39909=VERTEX_POINT('',#184859);
#39910=VERTEX_POINT('',#184861);
#39911=VERTEX_POINT('',#184863);
#39912=VERTEX_POINT('',#184865);
#39913=VERTEX_POINT('',#184867);
#39914=VERTEX_POINT('',#184869);
#39915=VERTEX_POINT('',#184871);
#39916=VERTEX_POINT('',#184875);
#39917=VERTEX_POINT('',#184876);
#39918=VERTEX_POINT('',#184878);
#39919=VERTEX_POINT('',#184880);
#39920=VERTEX_POINT('',#184882);
#39921=VERTEX_POINT('',#184884);
#39922=VERTEX_POINT('',#184886);
#39923=VERTEX_POINT('',#184888);
#39924=VERTEX_POINT('',#184890);
#39925=VERTEX_POINT('',#184892);
#39926=VERTEX_POINT('',#184894);
#39927=VERTEX_POINT('',#184896);
#39928=VERTEX_POINT('',#184900);
#39929=VERTEX_POINT('',#184901);
#39930=VERTEX_POINT('',#184903);
#39931=VERTEX_POINT('',#184905);
#39932=VERTEX_POINT('',#184909);
#39933=VERTEX_POINT('',#184910);
#39934=VERTEX_POINT('',#184912);
#39935=VERTEX_POINT('',#184914);
#39936=VERTEX_POINT('',#184916);
#39937=VERTEX_POINT('',#184918);
#39938=VERTEX_POINT('',#184920);
#39939=VERTEX_POINT('',#184922);
#39940=VERTEX_POINT('',#184924);
#39941=VERTEX_POINT('',#184926);
#39942=VERTEX_POINT('',#184928);
#39943=VERTEX_POINT('',#184930);
#39944=VERTEX_POINT('',#184934);
#39945=VERTEX_POINT('',#184935);
#39946=VERTEX_POINT('',#184937);
#39947=VERTEX_POINT('',#184939);
#39948=VERTEX_POINT('',#184941);
#39949=VERTEX_POINT('',#184943);
#39950=VERTEX_POINT('',#184945);
#39951=VERTEX_POINT('',#184947);
#39952=VERTEX_POINT('',#184949);
#39953=VERTEX_POINT('',#184951);
#39954=VERTEX_POINT('',#184953);
#39955=VERTEX_POINT('',#184955);
#39956=VERTEX_POINT('',#184959);
#39957=VERTEX_POINT('',#184960);
#39958=VERTEX_POINT('',#184962);
#39959=VERTEX_POINT('',#184964);
#39960=VERTEX_POINT('',#184968);
#39961=VERTEX_POINT('',#184969);
#39962=VERTEX_POINT('',#184971);
#39963=VERTEX_POINT('',#184973);
#39964=VERTEX_POINT('',#184975);
#39965=VERTEX_POINT('',#184977);
#39966=VERTEX_POINT('',#184979);
#39967=VERTEX_POINT('',#184981);
#39968=VERTEX_POINT('',#184983);
#39969=VERTEX_POINT('',#184985);
#39970=VERTEX_POINT('',#184987);
#39971=VERTEX_POINT('',#184989);
#39972=VERTEX_POINT('',#184993);
#39973=VERTEX_POINT('',#184994);
#39974=VERTEX_POINT('',#184996);
#39975=VERTEX_POINT('',#184998);
#39976=VERTEX_POINT('',#185000);
#39977=VERTEX_POINT('',#185002);
#39978=VERTEX_POINT('',#185004);
#39979=VERTEX_POINT('',#185006);
#39980=VERTEX_POINT('',#185008);
#39981=VERTEX_POINT('',#185010);
#39982=VERTEX_POINT('',#185012);
#39983=VERTEX_POINT('',#185014);
#39984=VERTEX_POINT('',#185018);
#39985=VERTEX_POINT('',#185019);
#39986=VERTEX_POINT('',#185021);
#39987=VERTEX_POINT('',#185023);
#39988=VERTEX_POINT('',#185027);
#39989=VERTEX_POINT('',#185028);
#39990=VERTEX_POINT('',#185030);
#39991=VERTEX_POINT('',#185032);
#39992=VERTEX_POINT('',#185034);
#39993=VERTEX_POINT('',#185036);
#39994=VERTEX_POINT('',#185038);
#39995=VERTEX_POINT('',#185040);
#39996=VERTEX_POINT('',#185042);
#39997=VERTEX_POINT('',#185044);
#39998=VERTEX_POINT('',#185046);
#39999=VERTEX_POINT('',#185048);
#40000=VERTEX_POINT('',#185052);
#40001=VERTEX_POINT('',#185053);
#40002=VERTEX_POINT('',#185055);
#40003=VERTEX_POINT('',#185057);
#40004=VERTEX_POINT('',#185059);
#40005=VERTEX_POINT('',#185061);
#40006=VERTEX_POINT('',#185063);
#40007=VERTEX_POINT('',#185065);
#40008=VERTEX_POINT('',#185067);
#40009=VERTEX_POINT('',#185069);
#40010=VERTEX_POINT('',#185071);
#40011=VERTEX_POINT('',#185073);
#40012=VERTEX_POINT('',#185080);
#40013=VERTEX_POINT('',#185081);
#40014=VERTEX_POINT('',#185083);
#40015=VERTEX_POINT('',#185085);
#40016=VERTEX_POINT('',#185087);
#40017=VERTEX_POINT('',#185089);
#40018=VERTEX_POINT('',#185091);
#40019=VERTEX_POINT('',#185093);
#40020=VERTEX_POINT('',#185095);
#40021=VERTEX_POINT('',#185097);
#40022=VERTEX_POINT('',#185099);
#40023=VERTEX_POINT('',#185101);
#40024=VERTEX_POINT('',#185105);
#40025=VERTEX_POINT('',#185106);
#40026=VERTEX_POINT('',#185108);
#40027=VERTEX_POINT('',#185110);
#40028=VERTEX_POINT('',#185112);
#40029=VERTEX_POINT('',#185114);
#40030=VERTEX_POINT('',#185116);
#40031=VERTEX_POINT('',#185118);
#40032=VERTEX_POINT('',#185120);
#40033=VERTEX_POINT('',#185122);
#40034=VERTEX_POINT('',#185124);
#40035=VERTEX_POINT('',#185126);
#40036=VERTEX_POINT('',#185130);
#40037=VERTEX_POINT('',#185131);
#40038=VERTEX_POINT('',#185133);
#40039=VERTEX_POINT('',#185135);
#40040=VERTEX_POINT('',#185139);
#40041=VERTEX_POINT('',#185140);
#40042=VERTEX_POINT('',#185142);
#40043=VERTEX_POINT('',#185144);
#40044=VERTEX_POINT('',#185146);
#40045=VERTEX_POINT('',#185148);
#40046=VERTEX_POINT('',#185150);
#40047=VERTEX_POINT('',#185152);
#40048=VERTEX_POINT('',#185154);
#40049=VERTEX_POINT('',#185156);
#40050=VERTEX_POINT('',#185158);
#40051=VERTEX_POINT('',#185160);
#40052=VERTEX_POINT('',#185164);
#40053=VERTEX_POINT('',#185165);
#40054=VERTEX_POINT('',#185167);
#40055=VERTEX_POINT('',#185169);
#40056=VERTEX_POINT('',#185171);
#40057=VERTEX_POINT('',#185173);
#40058=VERTEX_POINT('',#185175);
#40059=VERTEX_POINT('',#185177);
#40060=VERTEX_POINT('',#185179);
#40061=VERTEX_POINT('',#185181);
#40062=VERTEX_POINT('',#185183);
#40063=VERTEX_POINT('',#185185);
#40064=VERTEX_POINT('',#185189);
#40065=VERTEX_POINT('',#185190);
#40066=VERTEX_POINT('',#185192);
#40067=VERTEX_POINT('',#185194);
#40068=VERTEX_POINT('',#185198);
#40069=VERTEX_POINT('',#185199);
#40070=VERTEX_POINT('',#185201);
#40071=VERTEX_POINT('',#185203);
#40072=VERTEX_POINT('',#185205);
#40073=VERTEX_POINT('',#185207);
#40074=VERTEX_POINT('',#185209);
#40075=VERTEX_POINT('',#185211);
#40076=VERTEX_POINT('',#185213);
#40077=VERTEX_POINT('',#185215);
#40078=VERTEX_POINT('',#185217);
#40079=VERTEX_POINT('',#185219);
#40080=VERTEX_POINT('',#185223);
#40081=VERTEX_POINT('',#185224);
#40082=VERTEX_POINT('',#185226);
#40083=VERTEX_POINT('',#185228);
#40084=VERTEX_POINT('',#185230);
#40085=VERTEX_POINT('',#185232);
#40086=VERTEX_POINT('',#185234);
#40087=VERTEX_POINT('',#185236);
#40088=VERTEX_POINT('',#185238);
#40089=VERTEX_POINT('',#185240);
#40090=VERTEX_POINT('',#185242);
#40091=VERTEX_POINT('',#185244);
#40092=VERTEX_POINT('',#185248);
#40093=VERTEX_POINT('',#185249);
#40094=VERTEX_POINT('',#185251);
#40095=VERTEX_POINT('',#185253);
#40096=VERTEX_POINT('',#185257);
#40097=VERTEX_POINT('',#185258);
#40098=VERTEX_POINT('',#185260);
#40099=VERTEX_POINT('',#185262);
#40100=VERTEX_POINT('',#185264);
#40101=VERTEX_POINT('',#185266);
#40102=VERTEX_POINT('',#185268);
#40103=VERTEX_POINT('',#185270);
#40104=VERTEX_POINT('',#185272);
#40105=VERTEX_POINT('',#185274);
#40106=VERTEX_POINT('',#185276);
#40107=VERTEX_POINT('',#185278);
#40108=VERTEX_POINT('',#185282);
#40109=VERTEX_POINT('',#185283);
#40110=VERTEX_POINT('',#185285);
#40111=VERTEX_POINT('',#185287);
#40112=VERTEX_POINT('',#185289);
#40113=VERTEX_POINT('',#185291);
#40114=VERTEX_POINT('',#185293);
#40115=VERTEX_POINT('',#185295);
#40116=VERTEX_POINT('',#185297);
#40117=VERTEX_POINT('',#185299);
#40118=VERTEX_POINT('',#185301);
#40119=VERTEX_POINT('',#185303);
#40120=VERTEX_POINT('',#185307);
#40121=VERTEX_POINT('',#185308);
#40122=VERTEX_POINT('',#185310);
#40123=VERTEX_POINT('',#185312);
#40124=VERTEX_POINT('',#185316);
#40125=VERTEX_POINT('',#185317);
#40126=VERTEX_POINT('',#185319);
#40127=VERTEX_POINT('',#185321);
#40128=VERTEX_POINT('',#185323);
#40129=VERTEX_POINT('',#185325);
#40130=VERTEX_POINT('',#185327);
#40131=VERTEX_POINT('',#185329);
#40132=VERTEX_POINT('',#185331);
#40133=VERTEX_POINT('',#185333);
#40134=VERTEX_POINT('',#185335);
#40135=VERTEX_POINT('',#185337);
#40136=VERTEX_POINT('',#185341);
#40137=VERTEX_POINT('',#185342);
#40138=VERTEX_POINT('',#185344);
#40139=VERTEX_POINT('',#185346);
#40140=VERTEX_POINT('',#185348);
#40141=VERTEX_POINT('',#185350);
#40142=VERTEX_POINT('',#185352);
#40143=VERTEX_POINT('',#185354);
#40144=VERTEX_POINT('',#185356);
#40145=VERTEX_POINT('',#185358);
#40146=VERTEX_POINT('',#185360);
#40147=VERTEX_POINT('',#185362);
#40148=VERTEX_POINT('',#185366);
#40149=VERTEX_POINT('',#185367);
#40150=VERTEX_POINT('',#185369);
#40151=VERTEX_POINT('',#185371);
#40152=VERTEX_POINT('',#185375);
#40153=VERTEX_POINT('',#185376);
#40154=VERTEX_POINT('',#185378);
#40155=VERTEX_POINT('',#185380);
#40156=VERTEX_POINT('',#185382);
#40157=VERTEX_POINT('',#185384);
#40158=VERTEX_POINT('',#185386);
#40159=VERTEX_POINT('',#185388);
#40160=VERTEX_POINT('',#185390);
#40161=VERTEX_POINT('',#185392);
#40162=VERTEX_POINT('',#185394);
#40163=VERTEX_POINT('',#185396);
#40164=VERTEX_POINT('',#185400);
#40165=VERTEX_POINT('',#185401);
#40166=VERTEX_POINT('',#185403);
#40167=VERTEX_POINT('',#185405);
#40168=VERTEX_POINT('',#185407);
#40169=VERTEX_POINT('',#185409);
#40170=VERTEX_POINT('',#185411);
#40171=VERTEX_POINT('',#185413);
#40172=VERTEX_POINT('',#185415);
#40173=VERTEX_POINT('',#185417);
#40174=VERTEX_POINT('',#185419);
#40175=VERTEX_POINT('',#185421);
#40176=VERTEX_POINT('',#185425);
#40177=VERTEX_POINT('',#185426);
#40178=VERTEX_POINT('',#185428);
#40179=VERTEX_POINT('',#185430);
#40180=VERTEX_POINT('',#185434);
#40181=VERTEX_POINT('',#185435);
#40182=VERTEX_POINT('',#185437);
#40183=VERTEX_POINT('',#185439);
#40184=VERTEX_POINT('',#185441);
#40185=VERTEX_POINT('',#185443);
#40186=VERTEX_POINT('',#185445);
#40187=VERTEX_POINT('',#185447);
#40188=VERTEX_POINT('',#185449);
#40189=VERTEX_POINT('',#185451);
#40190=VERTEX_POINT('',#185453);
#40191=VERTEX_POINT('',#185455);
#40192=VERTEX_POINT('',#185459);
#40193=VERTEX_POINT('',#185460);
#40194=VERTEX_POINT('',#185462);
#40195=VERTEX_POINT('',#185464);
#40196=VERTEX_POINT('',#185466);
#40197=VERTEX_POINT('',#185468);
#40198=VERTEX_POINT('',#185470);
#40199=VERTEX_POINT('',#185472);
#40200=VERTEX_POINT('',#185474);
#40201=VERTEX_POINT('',#185476);
#40202=VERTEX_POINT('',#185478);
#40203=VERTEX_POINT('',#185480);
#40204=VERTEX_POINT('',#185484);
#40205=VERTEX_POINT('',#185485);
#40206=VERTEX_POINT('',#185487);
#40207=VERTEX_POINT('',#185489);
#40208=VERTEX_POINT('',#185493);
#40209=VERTEX_POINT('',#185494);
#40210=VERTEX_POINT('',#185496);
#40211=VERTEX_POINT('',#185498);
#40212=VERTEX_POINT('',#185500);
#40213=VERTEX_POINT('',#185502);
#40214=VERTEX_POINT('',#185504);
#40215=VERTEX_POINT('',#185506);
#40216=VERTEX_POINT('',#185508);
#40217=VERTEX_POINT('',#185510);
#40218=VERTEX_POINT('',#185512);
#40219=VERTEX_POINT('',#185514);
#40220=VERTEX_POINT('',#185518);
#40221=VERTEX_POINT('',#185519);
#40222=VERTEX_POINT('',#185521);
#40223=VERTEX_POINT('',#185523);
#40224=VERTEX_POINT('',#185525);
#40225=VERTEX_POINT('',#185527);
#40226=VERTEX_POINT('',#185529);
#40227=VERTEX_POINT('',#185531);
#40228=VERTEX_POINT('',#185533);
#40229=VERTEX_POINT('',#185535);
#40230=VERTEX_POINT('',#185537);
#40231=VERTEX_POINT('',#185539);
#40232=VERTEX_POINT('',#185543);
#40233=VERTEX_POINT('',#185544);
#40234=VERTEX_POINT('',#185546);
#40235=VERTEX_POINT('',#185548);
#40236=VERTEX_POINT('',#185552);
#40237=VERTEX_POINT('',#185553);
#40238=VERTEX_POINT('',#185555);
#40239=VERTEX_POINT('',#185557);
#40240=VERTEX_POINT('',#185559);
#40241=VERTEX_POINT('',#185561);
#40242=VERTEX_POINT('',#185563);
#40243=VERTEX_POINT('',#185565);
#40244=VERTEX_POINT('',#185567);
#40245=VERTEX_POINT('',#185569);
#40246=VERTEX_POINT('',#185571);
#40247=VERTEX_POINT('',#185573);
#40248=VERTEX_POINT('',#185577);
#40249=VERTEX_POINT('',#185578);
#40250=VERTEX_POINT('',#185580);
#40251=VERTEX_POINT('',#185582);
#40252=VERTEX_POINT('',#185584);
#40253=VERTEX_POINT('',#185586);
#40254=VERTEX_POINT('',#185588);
#40255=VERTEX_POINT('',#185590);
#40256=VERTEX_POINT('',#185592);
#40257=VERTEX_POINT('',#185594);
#40258=VERTEX_POINT('',#185596);
#40259=VERTEX_POINT('',#185598);
#40260=VERTEX_POINT('',#185602);
#40261=VERTEX_POINT('',#185603);
#40262=VERTEX_POINT('',#185605);
#40263=VERTEX_POINT('',#185607);
#40264=VERTEX_POINT('',#185611);
#40265=VERTEX_POINT('',#185612);
#40266=VERTEX_POINT('',#185614);
#40267=VERTEX_POINT('',#185616);
#40268=VERTEX_POINT('',#185618);
#40269=VERTEX_POINT('',#185620);
#40270=VERTEX_POINT('',#185622);
#40271=VERTEX_POINT('',#185624);
#40272=VERTEX_POINT('',#185626);
#40273=VERTEX_POINT('',#185628);
#40274=VERTEX_POINT('',#185630);
#40275=VERTEX_POINT('',#185632);
#40276=VERTEX_POINT('',#185636);
#40277=VERTEX_POINT('',#185637);
#40278=VERTEX_POINT('',#185639);
#40279=VERTEX_POINT('',#185641);
#40280=VERTEX_POINT('',#185643);
#40281=VERTEX_POINT('',#185645);
#40282=VERTEX_POINT('',#185647);
#40283=VERTEX_POINT('',#185649);
#40284=VERTEX_POINT('',#185651);
#40285=VERTEX_POINT('',#185653);
#40286=VERTEX_POINT('',#185655);
#40287=VERTEX_POINT('',#185657);
#40288=VERTEX_POINT('',#185661);
#40289=VERTEX_POINT('',#185662);
#40290=VERTEX_POINT('',#185664);
#40291=VERTEX_POINT('',#185666);
#40292=VERTEX_POINT('',#185670);
#40293=VERTEX_POINT('',#185671);
#40294=VERTEX_POINT('',#185673);
#40295=VERTEX_POINT('',#185675);
#40296=VERTEX_POINT('',#185677);
#40297=VERTEX_POINT('',#185679);
#40298=VERTEX_POINT('',#185681);
#40299=VERTEX_POINT('',#185683);
#40300=VERTEX_POINT('',#185685);
#40301=VERTEX_POINT('',#185687);
#40302=VERTEX_POINT('',#185689);
#40303=VERTEX_POINT('',#185691);
#40304=VERTEX_POINT('',#185695);
#40305=VERTEX_POINT('',#185696);
#40306=VERTEX_POINT('',#185698);
#40307=VERTEX_POINT('',#185700);
#40308=VERTEX_POINT('',#185702);
#40309=VERTEX_POINT('',#185704);
#40310=VERTEX_POINT('',#185706);
#40311=VERTEX_POINT('',#185708);
#40312=VERTEX_POINT('',#185710);
#40313=VERTEX_POINT('',#185712);
#40314=VERTEX_POINT('',#185714);
#40315=VERTEX_POINT('',#185716);
#40316=VERTEX_POINT('',#185720);
#40317=VERTEX_POINT('',#185721);
#40318=VERTEX_POINT('',#185723);
#40319=VERTEX_POINT('',#185725);
#40320=VERTEX_POINT('',#185729);
#40321=VERTEX_POINT('',#185730);
#40322=VERTEX_POINT('',#185732);
#40323=VERTEX_POINT('',#185734);
#40324=VERTEX_POINT('',#185736);
#40325=VERTEX_POINT('',#185738);
#40326=VERTEX_POINT('',#185740);
#40327=VERTEX_POINT('',#185742);
#40328=VERTEX_POINT('',#185744);
#40329=VERTEX_POINT('',#185746);
#40330=VERTEX_POINT('',#185748);
#40331=VERTEX_POINT('',#185750);
#40332=VERTEX_POINT('',#185754);
#40333=VERTEX_POINT('',#185755);
#40334=VERTEX_POINT('',#185757);
#40335=VERTEX_POINT('',#185759);
#40336=VERTEX_POINT('',#185761);
#40337=VERTEX_POINT('',#185763);
#40338=VERTEX_POINT('',#185765);
#40339=VERTEX_POINT('',#185767);
#40340=VERTEX_POINT('',#185769);
#40341=VERTEX_POINT('',#185771);
#40342=VERTEX_POINT('',#185773);
#40343=VERTEX_POINT('',#185775);
#40344=VERTEX_POINT('',#185779);
#40345=VERTEX_POINT('',#185780);
#40346=VERTEX_POINT('',#185782);
#40347=VERTEX_POINT('',#185784);
#40348=VERTEX_POINT('',#185788);
#40349=VERTEX_POINT('',#185789);
#40350=VERTEX_POINT('',#185791);
#40351=VERTEX_POINT('',#185793);
#40352=VERTEX_POINT('',#185795);
#40353=VERTEX_POINT('',#185797);
#40354=VERTEX_POINT('',#185799);
#40355=VERTEX_POINT('',#185801);
#40356=VERTEX_POINT('',#185803);
#40357=VERTEX_POINT('',#185805);
#40358=VERTEX_POINT('',#185807);
#40359=VERTEX_POINT('',#185809);
#40360=VERTEX_POINT('',#185813);
#40361=VERTEX_POINT('',#185814);
#40362=VERTEX_POINT('',#185816);
#40363=VERTEX_POINT('',#185818);
#40364=VERTEX_POINT('',#185820);
#40365=VERTEX_POINT('',#185822);
#40366=VERTEX_POINT('',#185824);
#40367=VERTEX_POINT('',#185826);
#40368=VERTEX_POINT('',#185828);
#40369=VERTEX_POINT('',#185830);
#40370=VERTEX_POINT('',#185832);
#40371=VERTEX_POINT('',#185834);
#40372=VERTEX_POINT('',#185838);
#40373=VERTEX_POINT('',#185839);
#40374=VERTEX_POINT('',#185841);
#40375=VERTEX_POINT('',#185843);
#40376=VERTEX_POINT('',#185847);
#40377=VERTEX_POINT('',#185848);
#40378=VERTEX_POINT('',#185850);
#40379=VERTEX_POINT('',#185852);
#40380=VERTEX_POINT('',#185854);
#40381=VERTEX_POINT('',#185856);
#40382=VERTEX_POINT('',#185858);
#40383=VERTEX_POINT('',#185860);
#40384=VERTEX_POINT('',#185862);
#40385=VERTEX_POINT('',#185864);
#40386=VERTEX_POINT('',#185866);
#40387=VERTEX_POINT('',#185868);
#40388=VERTEX_POINT('',#185872);
#40389=VERTEX_POINT('',#185873);
#40390=VERTEX_POINT('',#185875);
#40391=VERTEX_POINT('',#185877);
#40392=VERTEX_POINT('',#185879);
#40393=VERTEX_POINT('',#185881);
#40394=VERTEX_POINT('',#185883);
#40395=VERTEX_POINT('',#185885);
#40396=VERTEX_POINT('',#185887);
#40397=VERTEX_POINT('',#185889);
#40398=VERTEX_POINT('',#185891);
#40399=VERTEX_POINT('',#185893);
#40400=VERTEX_POINT('',#185897);
#40401=VERTEX_POINT('',#185898);
#40402=VERTEX_POINT('',#185900);
#40403=VERTEX_POINT('',#185902);
#40404=VERTEX_POINT('',#185906);
#40405=VERTEX_POINT('',#185907);
#40406=VERTEX_POINT('',#185909);
#40407=VERTEX_POINT('',#185911);
#40408=VERTEX_POINT('',#185913);
#40409=VERTEX_POINT('',#185915);
#40410=VERTEX_POINT('',#185917);
#40411=VERTEX_POINT('',#185919);
#40412=VERTEX_POINT('',#185921);
#40413=VERTEX_POINT('',#185923);
#40414=VERTEX_POINT('',#185925);
#40415=VERTEX_POINT('',#185927);
#40416=VERTEX_POINT('',#185931);
#40417=VERTEX_POINT('',#185932);
#40418=VERTEX_POINT('',#185934);
#40419=VERTEX_POINT('',#185936);
#40420=VERTEX_POINT('',#185938);
#40421=VERTEX_POINT('',#185940);
#40422=VERTEX_POINT('',#185942);
#40423=VERTEX_POINT('',#185944);
#40424=VERTEX_POINT('',#185946);
#40425=VERTEX_POINT('',#185948);
#40426=VERTEX_POINT('',#185950);
#40427=VERTEX_POINT('',#185952);
#40428=VERTEX_POINT('',#210488);
#40429=VERTEX_POINT('',#210489);
#40430=VERTEX_POINT('',#210491);
#40431=VERTEX_POINT('',#210493);
#40432=VERTEX_POINT('',#210497);
#40433=VERTEX_POINT('',#210498);
#40434=VERTEX_POINT('',#210500);
#40435=VERTEX_POINT('',#210502);
#40436=VERTEX_POINT('',#210506);
#40437=VERTEX_POINT('',#210507);
#40438=VERTEX_POINT('',#210509);
#40439=VERTEX_POINT('',#210511);
#40440=VERTEX_POINT('',#210515);
#40441=VERTEX_POINT('',#210516);
#40442=VERTEX_POINT('',#210518);
#40443=VERTEX_POINT('',#210520);
#40444=VERTEX_POINT('',#210522);
#40445=VERTEX_POINT('',#210526);
#40446=VERTEX_POINT('',#210528);
#40447=VERTEX_POINT('',#210530);
#40448=VERTEX_POINT('',#210534);
#40449=VERTEX_POINT('',#210536);
#40450=VERTEX_POINT('',#210540);
#40451=VERTEX_POINT('',#210542);
#40452=VERTEX_POINT('',#210544);
#40453=VERTEX_POINT('',#210548);
#40454=VERTEX_POINT('',#210550);
#40455=VERTEX_POINT('',#210554);
#40456=VERTEX_POINT('',#210556);
#40457=VERTEX_POINT('',#210562);
#40458=VERTEX_POINT('',#210563);
#40459=VERTEX_POINT('',#210565);
#40460=VERTEX_POINT('',#210609);
#40461=VERTEX_POINT('',#210611);
#40462=VERTEX_POINT('',#210613);
#40463=VERTEX_POINT('',#210615);
#40464=VERTEX_POINT('',#210656);
#40465=VERTEX_POINT('',#210658);
#40466=VERTEX_POINT('',#210702);
#40467=VERTEX_POINT('',#210704);
#40468=VERTEX_POINT('',#210706);
#40469=VERTEX_POINT('',#210708);
#40470=VERTEX_POINT('',#210749);
#40471=VERTEX_POINT('',#210751);
#40472=VERTEX_POINT('',#210795);
#40473=VERTEX_POINT('',#210797);
#40474=VERTEX_POINT('',#210799);
#40475=VERTEX_POINT('',#210801);
#40476=VERTEX_POINT('',#210842);
#40477=VERTEX_POINT('',#210844);
#40478=VERTEX_POINT('',#210888);
#40479=VERTEX_POINT('',#210890);
#40480=VERTEX_POINT('',#210892);
#40481=VERTEX_POINT('',#210894);
#40482=VERTEX_POINT('',#210935);
#40483=VERTEX_POINT('',#210937);
#40484=VERTEX_POINT('',#210981);
#40485=VERTEX_POINT('',#210983);
#40486=VERTEX_POINT('',#210985);
#40487=VERTEX_POINT('',#210987);
#40488=VERTEX_POINT('',#211028);
#40489=VERTEX_POINT('',#211030);
#40490=VERTEX_POINT('',#211074);
#40491=VERTEX_POINT('',#211076);
#40492=VERTEX_POINT('',#211078);
#40493=VERTEX_POINT('',#211080);
#40494=VERTEX_POINT('',#211121);
#40495=VERTEX_POINT('',#211123);
#40496=VERTEX_POINT('',#211167);
#40497=VERTEX_POINT('',#211169);
#40498=VERTEX_POINT('',#211171);
#40499=VERTEX_POINT('',#211173);
#40500=VERTEX_POINT('',#211214);
#40501=VERTEX_POINT('',#211216);
#40502=VERTEX_POINT('',#211260);
#40503=VERTEX_POINT('',#211262);
#40504=VERTEX_POINT('',#211264);
#40505=VERTEX_POINT('',#211266);
#40506=VERTEX_POINT('',#211307);
#40507=VERTEX_POINT('',#211309);
#40508=VERTEX_POINT('',#211353);
#40509=VERTEX_POINT('',#211355);
#40510=VERTEX_POINT('',#211357);
#40511=VERTEX_POINT('',#211359);
#40512=VERTEX_POINT('',#211400);
#40513=VERTEX_POINT('',#211402);
#40514=VERTEX_POINT('',#211446);
#40515=VERTEX_POINT('',#211448);
#40516=VERTEX_POINT('',#211450);
#40517=VERTEX_POINT('',#211452);
#40518=VERTEX_POINT('',#211493);
#40519=VERTEX_POINT('',#211495);
#40520=VERTEX_POINT('',#211539);
#40521=VERTEX_POINT('',#211541);
#40522=VERTEX_POINT('',#211543);
#40523=VERTEX_POINT('',#211545);
#40524=VERTEX_POINT('',#211586);
#40525=VERTEX_POINT('',#211588);
#40526=VERTEX_POINT('',#211632);
#40527=VERTEX_POINT('',#211634);
#40528=VERTEX_POINT('',#211636);
#40529=VERTEX_POINT('',#211638);
#40530=VERTEX_POINT('',#211679);
#40531=VERTEX_POINT('',#211681);
#40532=VERTEX_POINT('',#211725);
#40533=VERTEX_POINT('',#211727);
#40534=VERTEX_POINT('',#211729);
#40535=VERTEX_POINT('',#211731);
#40536=VERTEX_POINT('',#211772);
#40537=VERTEX_POINT('',#211774);
#40538=VERTEX_POINT('',#211818);
#40539=VERTEX_POINT('',#211820);
#40540=VERTEX_POINT('',#211822);
#40541=VERTEX_POINT('',#211824);
#40542=VERTEX_POINT('',#211865);
#40543=VERTEX_POINT('',#211867);
#40544=VERTEX_POINT('',#211911);
#40545=VERTEX_POINT('',#211913);
#40546=VERTEX_POINT('',#211915);
#40547=VERTEX_POINT('',#211917);
#40548=VERTEX_POINT('',#211958);
#40549=VERTEX_POINT('',#211960);
#40550=VERTEX_POINT('',#212004);
#40551=VERTEX_POINT('',#212006);
#40552=VERTEX_POINT('',#212008);
#40553=VERTEX_POINT('',#212010);
#40554=VERTEX_POINT('',#212051);
#40555=VERTEX_POINT('',#212053);
#40556=VERTEX_POINT('',#212097);
#40557=VERTEX_POINT('',#212099);
#40558=VERTEX_POINT('',#212101);
#40559=VERTEX_POINT('',#212103);
#40560=VERTEX_POINT('',#212144);
#40561=VERTEX_POINT('',#212146);
#40562=VERTEX_POINT('',#212190);
#40563=VERTEX_POINT('',#212192);
#40564=VERTEX_POINT('',#212194);
#40565=VERTEX_POINT('',#212196);
#40566=VERTEX_POINT('',#212237);
#40567=VERTEX_POINT('',#212239);
#40568=VERTEX_POINT('',#212283);
#40569=VERTEX_POINT('',#212285);
#40570=VERTEX_POINT('',#212287);
#40571=VERTEX_POINT('',#212289);
#40572=VERTEX_POINT('',#212330);
#40573=VERTEX_POINT('',#212332);
#40574=VERTEX_POINT('',#212376);
#40575=VERTEX_POINT('',#212378);
#40576=VERTEX_POINT('',#212380);
#40577=VERTEX_POINT('',#212382);
#40578=VERTEX_POINT('',#212423);
#40579=VERTEX_POINT('',#212425);
#40580=VERTEX_POINT('',#212469);
#40581=VERTEX_POINT('',#212471);
#40582=VERTEX_POINT('',#212473);
#40583=VERTEX_POINT('',#212475);
#40584=VERTEX_POINT('',#212516);
#40585=VERTEX_POINT('',#212518);
#40586=VERTEX_POINT('',#212562);
#40587=VERTEX_POINT('',#212564);
#40588=VERTEX_POINT('',#212566);
#40589=VERTEX_POINT('',#212568);
#40590=VERTEX_POINT('',#212609);
#40591=VERTEX_POINT('',#212611);
#40592=VERTEX_POINT('',#212655);
#40593=VERTEX_POINT('',#212657);
#40594=VERTEX_POINT('',#212659);
#40595=VERTEX_POINT('',#212661);
#40596=VERTEX_POINT('',#212702);
#40597=VERTEX_POINT('',#212704);
#40598=VERTEX_POINT('',#212748);
#40599=VERTEX_POINT('',#212750);
#40600=VERTEX_POINT('',#212752);
#40601=VERTEX_POINT('',#212754);
#40602=VERTEX_POINT('',#212795);
#40603=VERTEX_POINT('',#212797);
#40604=VERTEX_POINT('',#212841);
#40605=VERTEX_POINT('',#212843);
#40606=VERTEX_POINT('',#212845);
#40607=VERTEX_POINT('',#212847);
#40608=VERTEX_POINT('',#212888);
#40609=VERTEX_POINT('',#212890);
#40610=VERTEX_POINT('',#212934);
#40611=VERTEX_POINT('',#212936);
#40612=VERTEX_POINT('',#212938);
#40613=VERTEX_POINT('',#212940);
#40614=VERTEX_POINT('',#212981);
#40615=VERTEX_POINT('',#212983);
#40616=VERTEX_POINT('',#213027);
#40617=VERTEX_POINT('',#213029);
#40618=VERTEX_POINT('',#213031);
#40619=VERTEX_POINT('',#213033);
#40620=VERTEX_POINT('',#213074);
#40621=VERTEX_POINT('',#213076);
#40622=VERTEX_POINT('',#213120);
#40623=VERTEX_POINT('',#213122);
#40624=VERTEX_POINT('',#213124);
#40625=VERTEX_POINT('',#213126);
#40626=VERTEX_POINT('',#213167);
#40627=VERTEX_POINT('',#213169);
#40628=VERTEX_POINT('',#213213);
#40629=VERTEX_POINT('',#213215);
#40630=VERTEX_POINT('',#213217);
#40631=VERTEX_POINT('',#213219);
#40632=VERTEX_POINT('',#213260);
#40633=VERTEX_POINT('',#213262);
#40634=VERTEX_POINT('',#213306);
#40635=VERTEX_POINT('',#213308);
#40636=VERTEX_POINT('',#213310);
#40637=VERTEX_POINT('',#213353);
#40638=VERTEX_POINT('',#213397);
#40639=VERTEX_POINT('',#213399);
#40640=VERTEX_POINT('',#213401);
#40641=VERTEX_POINT('',#213403);
#40642=VERTEX_POINT('',#213444);
#40643=VERTEX_POINT('',#213446);
#40644=VERTEX_POINT('',#213490);
#40645=VERTEX_POINT('',#213492);
#40646=VERTEX_POINT('',#213494);
#40647=VERTEX_POINT('',#213496);
#40648=VERTEX_POINT('',#213537);
#40649=VERTEX_POINT('',#213539);
#40650=VERTEX_POINT('',#213583);
#40651=VERTEX_POINT('',#213585);
#40652=VERTEX_POINT('',#213587);
#40653=VERTEX_POINT('',#213589);
#40654=VERTEX_POINT('',#213630);
#40655=VERTEX_POINT('',#213632);
#40656=VERTEX_POINT('',#213676);
#40657=VERTEX_POINT('',#213678);
#40658=VERTEX_POINT('',#213680);
#40659=VERTEX_POINT('',#213682);
#40660=VERTEX_POINT('',#213723);
#40661=VERTEX_POINT('',#213725);
#40662=VERTEX_POINT('',#213769);
#40663=VERTEX_POINT('',#213771);
#40664=VERTEX_POINT('',#213773);
#40665=VERTEX_POINT('',#213775);
#40666=VERTEX_POINT('',#213816);
#40667=VERTEX_POINT('',#213818);
#40668=VERTEX_POINT('',#213862);
#40669=VERTEX_POINT('',#213864);
#40670=VERTEX_POINT('',#213866);
#40671=VERTEX_POINT('',#213868);
#40672=VERTEX_POINT('',#213909);
#40673=VERTEX_POINT('',#213911);
#40674=VERTEX_POINT('',#213955);
#40675=VERTEX_POINT('',#213957);
#40676=VERTEX_POINT('',#213959);
#40677=VERTEX_POINT('',#213961);
#40678=VERTEX_POINT('',#214002);
#40679=VERTEX_POINT('',#214004);
#40680=VERTEX_POINT('',#214048);
#40681=VERTEX_POINT('',#214050);
#40682=VERTEX_POINT('',#214052);
#40683=VERTEX_POINT('',#214054);
#40684=VERTEX_POINT('',#214095);
#40685=VERTEX_POINT('',#214097);
#40686=VERTEX_POINT('',#214141);
#40687=VERTEX_POINT('',#214143);
#40688=VERTEX_POINT('',#214145);
#40689=VERTEX_POINT('',#214147);
#40690=VERTEX_POINT('',#214188);
#40691=VERTEX_POINT('',#214190);
#40692=VERTEX_POINT('',#214234);
#40693=VERTEX_POINT('',#214236);
#40694=VERTEX_POINT('',#214238);
#40695=VERTEX_POINT('',#214240);
#40696=VERTEX_POINT('',#214281);
#40697=VERTEX_POINT('',#214283);
#40698=VERTEX_POINT('',#214327);
#40699=VERTEX_POINT('',#214329);
#40700=VERTEX_POINT('',#214331);
#40701=VERTEX_POINT('',#214333);
#40702=VERTEX_POINT('',#214374);
#40703=VERTEX_POINT('',#214376);
#40704=VERTEX_POINT('',#214420);
#40705=VERTEX_POINT('',#214422);
#40706=VERTEX_POINT('',#214424);
#40707=VERTEX_POINT('',#214426);
#40708=VERTEX_POINT('',#214467);
#40709=VERTEX_POINT('',#214469);
#40710=VERTEX_POINT('',#214513);
#40711=VERTEX_POINT('',#214515);
#40712=VERTEX_POINT('',#214517);
#40713=VERTEX_POINT('',#214519);
#40714=VERTEX_POINT('',#214560);
#40715=VERTEX_POINT('',#214562);
#40716=VERTEX_POINT('',#214606);
#40717=VERTEX_POINT('',#214608);
#40718=VERTEX_POINT('',#214610);
#40719=VERTEX_POINT('',#214612);
#40720=VERTEX_POINT('',#214653);
#40721=VERTEX_POINT('',#214655);
#40722=VERTEX_POINT('',#214699);
#40723=VERTEX_POINT('',#214701);
#40724=VERTEX_POINT('',#214703);
#40725=VERTEX_POINT('',#214745);
#40726=VERTEX_POINT('',#214789);
#40727=VERTEX_POINT('',#214791);
#40728=VERTEX_POINT('',#214793);
#40729=VERTEX_POINT('',#214795);
#40730=VERTEX_POINT('',#214836);
#40731=VERTEX_POINT('',#214838);
#40732=VERTEX_POINT('',#214882);
#40733=VERTEX_POINT('',#214884);
#40734=VERTEX_POINT('',#214886);
#40735=VERTEX_POINT('',#214888);
#40736=VERTEX_POINT('',#214929);
#40737=VERTEX_POINT('',#214931);
#40738=VERTEX_POINT('',#214975);
#40739=VERTEX_POINT('',#214977);
#40740=VERTEX_POINT('',#214979);
#40741=VERTEX_POINT('',#214981);
#40742=VERTEX_POINT('',#215022);
#40743=VERTEX_POINT('',#215024);
#40744=VERTEX_POINT('',#215068);
#40745=VERTEX_POINT('',#215070);
#40746=VERTEX_POINT('',#215072);
#40747=VERTEX_POINT('',#215074);
#40748=VERTEX_POINT('',#215115);
#40749=VERTEX_POINT('',#215117);
#40750=VERTEX_POINT('',#215161);
#40751=VERTEX_POINT('',#215163);
#40752=VERTEX_POINT('',#215165);
#40753=VERTEX_POINT('',#215167);
#40754=VERTEX_POINT('',#215208);
#40755=VERTEX_POINT('',#215210);
#40756=VERTEX_POINT('',#215254);
#40757=VERTEX_POINT('',#215256);
#40758=VERTEX_POINT('',#215258);
#40759=VERTEX_POINT('',#215260);
#40760=VERTEX_POINT('',#215301);
#40761=VERTEX_POINT('',#215303);
#40762=VERTEX_POINT('',#215347);
#40763=VERTEX_POINT('',#215349);
#40764=VERTEX_POINT('',#215351);
#40765=VERTEX_POINT('',#215353);
#40766=VERTEX_POINT('',#215394);
#40767=VERTEX_POINT('',#215396);
#40768=VERTEX_POINT('',#215440);
#40769=VERTEX_POINT('',#215442);
#40770=VERTEX_POINT('',#215444);
#40771=VERTEX_POINT('',#215446);
#40772=VERTEX_POINT('',#215487);
#40773=VERTEX_POINT('',#215489);
#40774=VERTEX_POINT('',#215533);
#40775=VERTEX_POINT('',#215535);
#40776=VERTEX_POINT('',#215537);
#40777=VERTEX_POINT('',#215539);
#40778=VERTEX_POINT('',#215580);
#40779=VERTEX_POINT('',#215582);
#40780=VERTEX_POINT('',#215626);
#40781=VERTEX_POINT('',#215628);
#40782=VERTEX_POINT('',#215630);
#40783=VERTEX_POINT('',#215632);
#40784=VERTEX_POINT('',#215673);
#40785=VERTEX_POINT('',#215675);
#40786=VERTEX_POINT('',#215719);
#40787=VERTEX_POINT('',#215721);
#40788=VERTEX_POINT('',#215723);
#40789=VERTEX_POINT('',#215725);
#40790=VERTEX_POINT('',#215766);
#40791=VERTEX_POINT('',#215768);
#40792=VERTEX_POINT('',#215812);
#40793=VERTEX_POINT('',#215814);
#40794=VERTEX_POINT('',#215816);
#40795=VERTEX_POINT('',#215818);
#40796=VERTEX_POINT('',#215859);
#40797=VERTEX_POINT('',#215861);
#40798=VERTEX_POINT('',#215905);
#40799=VERTEX_POINT('',#215907);
#40800=VERTEX_POINT('',#215909);
#40801=VERTEX_POINT('',#215911);
#40802=VERTEX_POINT('',#215952);
#40803=VERTEX_POINT('',#215954);
#40804=VERTEX_POINT('',#215998);
#40805=VERTEX_POINT('',#216000);
#40806=VERTEX_POINT('',#216002);
#40807=VERTEX_POINT('',#216004);
#40808=VERTEX_POINT('',#216045);
#40809=VERTEX_POINT('',#216047);
#40810=VERTEX_POINT('',#216091);
#40811=VERTEX_POINT('',#216093);
#40812=VERTEX_POINT('',#216095);
#40813=VERTEX_POINT('',#216138);
#40814=VERTEX_POINT('',#216176);
#40815=VERTEX_POINT('',#216178);
#40816=VERTEX_POINT('',#216180);
#40817=VERTEX_POINT('',#216182);
#40818=VERTEX_POINT('',#216223);
#40819=VERTEX_POINT('',#216225);
#40820=VERTEX_POINT('',#216263);
#40821=VERTEX_POINT('',#216265);
#40822=VERTEX_POINT('',#216267);
#40823=VERTEX_POINT('',#216269);
#40824=VERTEX_POINT('',#216310);
#40825=VERTEX_POINT('',#216312);
#40826=VERTEX_POINT('',#216350);
#40827=VERTEX_POINT('',#216352);
#40828=VERTEX_POINT('',#216354);
#40829=VERTEX_POINT('',#216356);
#40830=VERTEX_POINT('',#216397);
#40831=VERTEX_POINT('',#216399);
#40832=VERTEX_POINT('',#216437);
#40833=VERTEX_POINT('',#216439);
#40834=VERTEX_POINT('',#216441);
#40835=VERTEX_POINT('',#216443);
#40836=VERTEX_POINT('',#216484);
#40837=VERTEX_POINT('',#216486);
#40838=VERTEX_POINT('',#216524);
#40839=VERTEX_POINT('',#216526);
#40840=VERTEX_POINT('',#216528);
#40841=VERTEX_POINT('',#216530);
#40842=VERTEX_POINT('',#216571);
#40843=VERTEX_POINT('',#216573);
#40844=VERTEX_POINT('',#216611);
#40845=VERTEX_POINT('',#216613);
#40846=VERTEX_POINT('',#216615);
#40847=VERTEX_POINT('',#216617);
#40848=VERTEX_POINT('',#216658);
#40849=VERTEX_POINT('',#216660);
#40850=VERTEX_POINT('',#216698);
#40851=VERTEX_POINT('',#216700);
#40852=VERTEX_POINT('',#216702);
#40853=VERTEX_POINT('',#216704);
#40854=VERTEX_POINT('',#216745);
#40855=VERTEX_POINT('',#216747);
#40856=VERTEX_POINT('',#216785);
#40857=VERTEX_POINT('',#216787);
#40858=VERTEX_POINT('',#216789);
#40859=VERTEX_POINT('',#216791);
#40860=VERTEX_POINT('',#216832);
#40861=VERTEX_POINT('',#216834);
#40862=VERTEX_POINT('',#216872);
#40863=VERTEX_POINT('',#216874);
#40864=VERTEX_POINT('',#216876);
#40865=VERTEX_POINT('',#216878);
#40866=VERTEX_POINT('',#216919);
#40867=VERTEX_POINT('',#216921);
#40868=VERTEX_POINT('',#216959);
#40869=VERTEX_POINT('',#216961);
#40870=VERTEX_POINT('',#216963);
#40871=VERTEX_POINT('',#216965);
#40872=VERTEX_POINT('',#217006);
#40873=VERTEX_POINT('',#217008);
#40874=VERTEX_POINT('',#217046);
#40875=VERTEX_POINT('',#217048);
#40876=VERTEX_POINT('',#217050);
#40877=VERTEX_POINT('',#217052);
#40878=VERTEX_POINT('',#217093);
#40879=VERTEX_POINT('',#217095);
#40880=VERTEX_POINT('',#217133);
#40881=VERTEX_POINT('',#217135);
#40882=VERTEX_POINT('',#217137);
#40883=VERTEX_POINT('',#217139);
#40884=VERTEX_POINT('',#217180);
#40885=VERTEX_POINT('',#217182);
#40886=VERTEX_POINT('',#217220);
#40887=VERTEX_POINT('',#217222);
#40888=VERTEX_POINT('',#217224);
#40889=VERTEX_POINT('',#217226);
#40890=VERTEX_POINT('',#217267);
#40891=VERTEX_POINT('',#217269);
#40892=VERTEX_POINT('',#217307);
#40893=VERTEX_POINT('',#217309);
#40894=VERTEX_POINT('',#217311);
#40895=VERTEX_POINT('',#217313);
#40896=VERTEX_POINT('',#217354);
#40897=VERTEX_POINT('',#217356);
#40898=VERTEX_POINT('',#217394);
#40899=VERTEX_POINT('',#217396);
#40900=VERTEX_POINT('',#217398);
#40901=VERTEX_POINT('',#217400);
#40902=VERTEX_POINT('',#217441);
#40903=VERTEX_POINT('',#217443);
#40904=VERTEX_POINT('',#217481);
#40905=VERTEX_POINT('',#217483);
#40906=VERTEX_POINT('',#217485);
#40907=VERTEX_POINT('',#217487);
#40908=VERTEX_POINT('',#217528);
#40909=VERTEX_POINT('',#217530);
#40910=VERTEX_POINT('',#217568);
#40911=VERTEX_POINT('',#217570);
#40912=VERTEX_POINT('',#217572);
#40913=VERTEX_POINT('',#217574);
#40914=VERTEX_POINT('',#217615);
#40915=VERTEX_POINT('',#217617);
#40916=VERTEX_POINT('',#217655);
#40917=VERTEX_POINT('',#217657);
#40918=VERTEX_POINT('',#217659);
#40919=VERTEX_POINT('',#217661);
#40920=VERTEX_POINT('',#217702);
#40921=VERTEX_POINT('',#217704);
#40922=VERTEX_POINT('',#217742);
#40923=VERTEX_POINT('',#217744);
#40924=VERTEX_POINT('',#217746);
#40925=VERTEX_POINT('',#217748);
#40926=VERTEX_POINT('',#217789);
#40927=VERTEX_POINT('',#217791);
#40928=VERTEX_POINT('',#217829);
#40929=VERTEX_POINT('',#217831);
#40930=VERTEX_POINT('',#217833);
#40931=VERTEX_POINT('',#217835);
#40932=VERTEX_POINT('',#217876);
#40933=VERTEX_POINT('',#217878);
#40934=VERTEX_POINT('',#217916);
#40935=VERTEX_POINT('',#217918);
#40936=VERTEX_POINT('',#217920);
#40937=VERTEX_POINT('',#217922);
#40938=VERTEX_POINT('',#217963);
#40939=VERTEX_POINT('',#217965);
#40940=VERTEX_POINT('',#218003);
#40941=VERTEX_POINT('',#218005);
#40942=VERTEX_POINT('',#218007);
#40943=VERTEX_POINT('',#218009);
#40944=VERTEX_POINT('',#218050);
#40945=VERTEX_POINT('',#218052);
#40946=VERTEX_POINT('',#218090);
#40947=VERTEX_POINT('',#218092);
#40948=VERTEX_POINT('',#218094);
#40949=VERTEX_POINT('',#218096);
#40950=VERTEX_POINT('',#218137);
#40951=VERTEX_POINT('',#218139);
#40952=VERTEX_POINT('',#218177);
#40953=VERTEX_POINT('',#218179);
#40954=VERTEX_POINT('',#218181);
#40955=VERTEX_POINT('',#218183);
#40956=VERTEX_POINT('',#218224);
#40957=VERTEX_POINT('',#218226);
#40958=VERTEX_POINT('',#218264);
#40959=VERTEX_POINT('',#218266);
#40960=VERTEX_POINT('',#218268);
#40961=VERTEX_POINT('',#218270);
#40962=VERTEX_POINT('',#218311);
#40963=VERTEX_POINT('',#218313);
#40964=VERTEX_POINT('',#218351);
#40965=VERTEX_POINT('',#218353);
#40966=VERTEX_POINT('',#218355);
#40967=VERTEX_POINT('',#218357);
#40968=VERTEX_POINT('',#218398);
#40969=VERTEX_POINT('',#218400);
#40970=VERTEX_POINT('',#218438);
#40971=VERTEX_POINT('',#218440);
#40972=VERTEX_POINT('',#218442);
#40973=VERTEX_POINT('',#218444);
#40974=VERTEX_POINT('',#218485);
#40975=VERTEX_POINT('',#218487);
#40976=VERTEX_POINT('',#218525);
#40977=VERTEX_POINT('',#218527);
#40978=VERTEX_POINT('',#218529);
#40979=VERTEX_POINT('',#218531);
#40980=VERTEX_POINT('',#218572);
#40981=VERTEX_POINT('',#218574);
#40982=VERTEX_POINT('',#218612);
#40983=VERTEX_POINT('',#218614);
#40984=VERTEX_POINT('',#218616);
#40985=VERTEX_POINT('',#218618);
#40986=VERTEX_POINT('',#218659);
#40987=VERTEX_POINT('',#218661);
#40988=VERTEX_POINT('',#218699);
#40989=VERTEX_POINT('',#218701);
#40990=VERTEX_POINT('',#218703);
#40991=VERTEX_POINT('',#218705);
#40992=VERTEX_POINT('',#218746);
#40993=VERTEX_POINT('',#218749);
#40994=VERTEX_POINT('',#218751);
#40995=VERTEX_POINT('',#218789);
#40996=VERTEX_POINT('',#218791);
#40997=VERTEX_POINT('',#218793);
#40998=VERTEX_POINT('',#218795);
#40999=VERTEX_POINT('',#218836);
#41000=VERTEX_POINT('',#218838);
#41001=VERTEX_POINT('',#218876);
#41002=VERTEX_POINT('',#218878);
#41003=VERTEX_POINT('',#218880);
#41004=VERTEX_POINT('',#218882);
#41005=VERTEX_POINT('',#218923);
#41006=VERTEX_POINT('',#218925);
#41007=VERTEX_POINT('',#218963);
#41008=VERTEX_POINT('',#218965);
#41009=VERTEX_POINT('',#218967);
#41010=VERTEX_POINT('',#218969);
#41011=VERTEX_POINT('',#219010);
#41012=VERTEX_POINT('',#219012);
#41013=VERTEX_POINT('',#219050);
#41014=VERTEX_POINT('',#219052);
#41015=VERTEX_POINT('',#219054);
#41016=VERTEX_POINT('',#219056);
#41017=VERTEX_POINT('',#219097);
#41018=VERTEX_POINT('',#219099);
#41019=VERTEX_POINT('',#219137);
#41020=VERTEX_POINT('',#219139);
#41021=VERTEX_POINT('',#219141);
#41022=VERTEX_POINT('',#219143);
#41023=VERTEX_POINT('',#219184);
#41024=VERTEX_POINT('',#219186);
#41025=VERTEX_POINT('',#219224);
#41026=VERTEX_POINT('',#219226);
#41027=VERTEX_POINT('',#219228);
#41028=VERTEX_POINT('',#219230);
#41029=VERTEX_POINT('',#219271);
#41030=VERTEX_POINT('',#219273);
#41031=VERTEX_POINT('',#219311);
#41032=VERTEX_POINT('',#219313);
#41033=VERTEX_POINT('',#219315);
#41034=VERTEX_POINT('',#219317);
#41035=VERTEX_POINT('',#219358);
#41036=VERTEX_POINT('',#219360);
#41037=VERTEX_POINT('',#219398);
#41038=VERTEX_POINT('',#219400);
#41039=VERTEX_POINT('',#219402);
#41040=VERTEX_POINT('',#219404);
#41041=VERTEX_POINT('',#219445);
#41042=VERTEX_POINT('',#219447);
#41043=VERTEX_POINT('',#219485);
#41044=VERTEX_POINT('',#219487);
#41045=VERTEX_POINT('',#219489);
#41046=VERTEX_POINT('',#219491);
#41047=VERTEX_POINT('',#219532);
#41048=VERTEX_POINT('',#219534);
#41049=VERTEX_POINT('',#219572);
#41050=VERTEX_POINT('',#219574);
#41051=VERTEX_POINT('',#219576);
#41052=VERTEX_POINT('',#219578);
#41053=VERTEX_POINT('',#219619);
#41054=VERTEX_POINT('',#219621);
#41055=VERTEX_POINT('',#219659);
#41056=VERTEX_POINT('',#219661);
#41057=VERTEX_POINT('',#219663);
#41058=VERTEX_POINT('',#219665);
#41059=VERTEX_POINT('',#219706);
#41060=VERTEX_POINT('',#219708);
#41061=VERTEX_POINT('',#219746);
#41062=VERTEX_POINT('',#219748);
#41063=VERTEX_POINT('',#219750);
#41064=VERTEX_POINT('',#219752);
#41065=VERTEX_POINT('',#219793);
#41066=VERTEX_POINT('',#219795);
#41067=VERTEX_POINT('',#219833);
#41068=VERTEX_POINT('',#219835);
#41069=VERTEX_POINT('',#219837);
#41070=VERTEX_POINT('',#219839);
#41071=VERTEX_POINT('',#219880);
#41072=VERTEX_POINT('',#219882);
#41073=VERTEX_POINT('',#219920);
#41074=VERTEX_POINT('',#219922);
#41075=VERTEX_POINT('',#219924);
#41076=VERTEX_POINT('',#219926);
#41077=VERTEX_POINT('',#219967);
#41078=VERTEX_POINT('',#219969);
#41079=VERTEX_POINT('',#220007);
#41080=VERTEX_POINT('',#220009);
#41081=VERTEX_POINT('',#220011);
#41082=VERTEX_POINT('',#220053);
#41083=VERTEX_POINT('',#220091);
#41084=VERTEX_POINT('',#220093);
#41085=VERTEX_POINT('',#220095);
#41086=VERTEX_POINT('',#220097);
#41087=VERTEX_POINT('',#220138);
#41088=VERTEX_POINT('',#220140);
#41089=VERTEX_POINT('',#220178);
#41090=VERTEX_POINT('',#220180);
#41091=VERTEX_POINT('',#220182);
#41092=VERTEX_POINT('',#220184);
#41093=VERTEX_POINT('',#220225);
#41094=VERTEX_POINT('',#220227);
#41095=VERTEX_POINT('',#220265);
#41096=VERTEX_POINT('',#220267);
#41097=VERTEX_POINT('',#220269);
#41098=VERTEX_POINT('',#220271);
#41099=VERTEX_POINT('',#220312);
#41100=VERTEX_POINT('',#220314);
#41101=VERTEX_POINT('',#220352);
#41102=VERTEX_POINT('',#220354);
#41103=VERTEX_POINT('',#220356);
#41104=VERTEX_POINT('',#220358);
#41105=VERTEX_POINT('',#220399);
#41106=VERTEX_POINT('',#220401);
#41107=VERTEX_POINT('',#220439);
#41108=VERTEX_POINT('',#220441);
#41109=VERTEX_POINT('',#220443);
#41110=VERTEX_POINT('',#220445);
#41111=VERTEX_POINT('',#220486);
#41112=VERTEX_POINT('',#220488);
#41113=VERTEX_POINT('',#220526);
#41114=VERTEX_POINT('',#220528);
#41115=VERTEX_POINT('',#220530);
#41116=VERTEX_POINT('',#220532);
#41117=VERTEX_POINT('',#220573);
#41118=VERTEX_POINT('',#220575);
#41119=VERTEX_POINT('',#220613);
#41120=VERTEX_POINT('',#220615);
#41121=VERTEX_POINT('',#220617);
#41122=VERTEX_POINT('',#220619);
#41123=VERTEX_POINT('',#220660);
#41124=VERTEX_POINT('',#220662);
#41125=VERTEX_POINT('',#220700);
#41126=VERTEX_POINT('',#220702);
#41127=VERTEX_POINT('',#220704);
#41128=VERTEX_POINT('',#220706);
#41129=VERTEX_POINT('',#220747);
#41130=VERTEX_POINT('',#220749);
#41131=VERTEX_POINT('',#220787);
#41132=VERTEX_POINT('',#220789);
#41133=VERTEX_POINT('',#220791);
#41134=VERTEX_POINT('',#220793);
#41135=VERTEX_POINT('',#220834);
#41136=VERTEX_POINT('',#220836);
#41137=VERTEX_POINT('',#220874);
#41138=VERTEX_POINT('',#220876);
#41139=VERTEX_POINT('',#220878);
#41140=VERTEX_POINT('',#220880);
#41141=VERTEX_POINT('',#220921);
#41142=VERTEX_POINT('',#220923);
#41143=VERTEX_POINT('',#220961);
#41144=VERTEX_POINT('',#220963);
#41145=VERTEX_POINT('',#220965);
#41146=VERTEX_POINT('',#220967);
#41147=VERTEX_POINT('',#221008);
#41148=VERTEX_POINT('',#221010);
#41149=VERTEX_POINT('',#221048);
#41150=VERTEX_POINT('',#221050);
#41151=VERTEX_POINT('',#221052);
#41152=VERTEX_POINT('',#221054);
#41153=VERTEX_POINT('',#221095);
#41154=VERTEX_POINT('',#221097);
#41155=VERTEX_POINT('',#221135);
#41156=VERTEX_POINT('',#221137);
#41157=VERTEX_POINT('',#221139);
#41158=VERTEX_POINT('',#221141);
#41159=VERTEX_POINT('',#221182);
#41160=VERTEX_POINT('',#221184);
#41161=VERTEX_POINT('',#221222);
#41162=VERTEX_POINT('',#221224);
#41163=VERTEX_POINT('',#221226);
#41164=VERTEX_POINT('',#221228);
#41165=VERTEX_POINT('',#221269);
#41166=VERTEX_POINT('',#221271);
#41167=VERTEX_POINT('',#221309);
#41168=VERTEX_POINT('',#221311);
#41169=VERTEX_POINT('',#221313);
#41170=VERTEX_POINT('',#221356);
#41171=VERTEX_POINT('',#221357);
#41172=VERTEX_POINT('',#221362);
#41173=VERTEX_POINT('',#221366);
#41174=VERTEX_POINT('',#221367);
#41175=VERTEX_POINT('',#221369);
#41176=VERTEX_POINT('',#221371);
#41177=VERTEX_POINT('',#221373);
#41178=VERTEX_POINT('',#221375);
#41179=VERTEX_POINT('',#221379);
#41180=VERTEX_POINT('',#221380);
#41181=VERTEX_POINT('',#221385);
#41182=VERTEX_POINT('',#221386);
#41183=VERTEX_POINT('',#221388);
#41184=VERTEX_POINT('',#221390);
#41185=VERTEX_POINT('',#221394);
#41186=VERTEX_POINT('',#221395);
#41187=VERTEX_POINT('',#221397);
#41188=VERTEX_POINT('',#221399);
#41189=VERTEX_POINT('',#221401);
#41190=VERTEX_POINT('',#221403);
#41191=VERTEX_POINT('',#221407);
#41192=VERTEX_POINT('',#221408);
#41193=VERTEX_POINT('',#221425);
#41194=VERTEX_POINT('',#221426);
#41195=VERTEX_POINT('',#221428);
#41196=VERTEX_POINT('',#221430);
#41197=VERTEX_POINT('',#221432);
#41198=VERTEX_POINT('',#221434);
#41199=VERTEX_POINT('',#221438);
#41200=VERTEX_POINT('',#221440);
#41201=VERTEX_POINT('',#221444);
#41202=VERTEX_POINT('',#221445);
#41203=VERTEX_POINT('',#221447);
#41204=VERTEX_POINT('',#221449);
#41205=VERTEX_POINT('',#221453);
#41206=VERTEX_POINT('',#221454);
#41207=VERTEX_POINT('',#221456);
#41208=VERTEX_POINT('',#221458);
#41209=VERTEX_POINT('',#221460);
#41210=VERTEX_POINT('',#221462);
#41211=VERTEX_POINT('',#221466);
#41212=VERTEX_POINT('',#221468);
#41213=VERTEX_POINT('',#221484);
#41214=VERTEX_POINT('',#221485);
#41215=VERTEX_POINT('',#221487);
#41216=VERTEX_POINT('',#221489);
#41217=VERTEX_POINT('',#221491);
#41218=VERTEX_POINT('',#221493);
#41219=VERTEX_POINT('',#221497);
#41220=VERTEX_POINT('',#221499);
#41221=VERTEX_POINT('',#221503);
#41222=VERTEX_POINT('',#221504);
#41223=VERTEX_POINT('',#221506);
#41224=VERTEX_POINT('',#221508);
#41225=VERTEX_POINT('',#221512);
#41226=VERTEX_POINT('',#221513);
#41227=VERTEX_POINT('',#221515);
#41228=VERTEX_POINT('',#221517);
#41229=VERTEX_POINT('',#221519);
#41230=VERTEX_POINT('',#221521);
#41231=VERTEX_POINT('',#221525);
#41232=VERTEX_POINT('',#221527);
#41233=VERTEX_POINT('',#221543);
#41234=VERTEX_POINT('',#221544);
#41235=VERTEX_POINT('',#221546);
#41236=VERTEX_POINT('',#221548);
#41237=VERTEX_POINT('',#221550);
#41238=VERTEX_POINT('',#221552);
#41239=VERTEX_POINT('',#221556);
#41240=VERTEX_POINT('',#221558);
#41241=VERTEX_POINT('',#221562);
#41242=VERTEX_POINT('',#221563);
#41243=VERTEX_POINT('',#221565);
#41244=VERTEX_POINT('',#221567);
#41245=VERTEX_POINT('',#221571);
#41246=VERTEX_POINT('',#221572);
#41247=VERTEX_POINT('',#221574);
#41248=VERTEX_POINT('',#221576);
#41249=VERTEX_POINT('',#221578);
#41250=VERTEX_POINT('',#221580);
#41251=VERTEX_POINT('',#221584);
#41252=VERTEX_POINT('',#221586);
#41253=VERTEX_POINT('',#221602);
#41254=VERTEX_POINT('',#221603);
#41255=VERTEX_POINT('',#221605);
#41256=VERTEX_POINT('',#221607);
#41257=VERTEX_POINT('',#221609);
#41258=VERTEX_POINT('',#221611);
#41259=VERTEX_POINT('',#221615);
#41260=VERTEX_POINT('',#221617);
#41261=VERTEX_POINT('',#221621);
#41262=VERTEX_POINT('',#221622);
#41263=VERTEX_POINT('',#221624);
#41264=VERTEX_POINT('',#221626);
#41265=VERTEX_POINT('',#221630);
#41266=VERTEX_POINT('',#221631);
#41267=VERTEX_POINT('',#221633);
#41268=VERTEX_POINT('',#221635);
#41269=VERTEX_POINT('',#221637);
#41270=VERTEX_POINT('',#221639);
#41271=VERTEX_POINT('',#221643);
#41272=VERTEX_POINT('',#221645);
#41273=VERTEX_POINT('',#221661);
#41274=VERTEX_POINT('',#221662);
#41275=VERTEX_POINT('',#221664);
#41276=VERTEX_POINT('',#221666);
#41277=VERTEX_POINT('',#221668);
#41278=VERTEX_POINT('',#221670);
#41279=VERTEX_POINT('',#221674);
#41280=VERTEX_POINT('',#221676);
#41281=VERTEX_POINT('',#221680);
#41282=VERTEX_POINT('',#221681);
#41283=VERTEX_POINT('',#221683);
#41284=VERTEX_POINT('',#221685);
#41285=VERTEX_POINT('',#221689);
#41286=VERTEX_POINT('',#221690);
#41287=VERTEX_POINT('',#221692);
#41288=VERTEX_POINT('',#221694);
#41289=VERTEX_POINT('',#221696);
#41290=VERTEX_POINT('',#221698);
#41291=VERTEX_POINT('',#221702);
#41292=VERTEX_POINT('',#221704);
#41293=VERTEX_POINT('',#221720);
#41294=VERTEX_POINT('',#221721);
#41295=VERTEX_POINT('',#221723);
#41296=VERTEX_POINT('',#221725);
#41297=VERTEX_POINT('',#221727);
#41298=VERTEX_POINT('',#221729);
#41299=VERTEX_POINT('',#221733);
#41300=VERTEX_POINT('',#221735);
#41301=VERTEX_POINT('',#221739);
#41302=VERTEX_POINT('',#221740);
#41303=VERTEX_POINT('',#221742);
#41304=VERTEX_POINT('',#221744);
#41305=VERTEX_POINT('',#221748);
#41306=VERTEX_POINT('',#221749);
#41307=VERTEX_POINT('',#221751);
#41308=VERTEX_POINT('',#221753);
#41309=VERTEX_POINT('',#221755);
#41310=VERTEX_POINT('',#221757);
#41311=VERTEX_POINT('',#221761);
#41312=VERTEX_POINT('',#221763);
#41313=VERTEX_POINT('',#221779);
#41314=VERTEX_POINT('',#221780);
#41315=VERTEX_POINT('',#221782);
#41316=VERTEX_POINT('',#221784);
#41317=VERTEX_POINT('',#221786);
#41318=VERTEX_POINT('',#221788);
#41319=VERTEX_POINT('',#221792);
#41320=VERTEX_POINT('',#221794);
#41321=VERTEX_POINT('',#221798);
#41322=VERTEX_POINT('',#221799);
#41323=VERTEX_POINT('',#221801);
#41324=VERTEX_POINT('',#221803);
#41325=VERTEX_POINT('',#221807);
#41326=VERTEX_POINT('',#221808);
#41327=VERTEX_POINT('',#221810);
#41328=VERTEX_POINT('',#221812);
#41329=VERTEX_POINT('',#221814);
#41330=VERTEX_POINT('',#221816);
#41331=VERTEX_POINT('',#221820);
#41332=VERTEX_POINT('',#221822);
#41333=VERTEX_POINT('',#221838);
#41334=VERTEX_POINT('',#221839);
#41335=VERTEX_POINT('',#221841);
#41336=VERTEX_POINT('',#221843);
#41337=VERTEX_POINT('',#221845);
#41338=VERTEX_POINT('',#221847);
#41339=VERTEX_POINT('',#221851);
#41340=VERTEX_POINT('',#221853);
#41341=VERTEX_POINT('',#221857);
#41342=VERTEX_POINT('',#221858);
#41343=VERTEX_POINT('',#221860);
#41344=VERTEX_POINT('',#221862);
#41345=VERTEX_POINT('',#221866);
#41346=VERTEX_POINT('',#221867);
#41347=VERTEX_POINT('',#221869);
#41348=VERTEX_POINT('',#221871);
#41349=VERTEX_POINT('',#221873);
#41350=VERTEX_POINT('',#221875);
#41351=VERTEX_POINT('',#221879);
#41352=VERTEX_POINT('',#221881);
#41353=VERTEX_POINT('',#221897);
#41354=VERTEX_POINT('',#221898);
#41355=VERTEX_POINT('',#221900);
#41356=VERTEX_POINT('',#221902);
#41357=VERTEX_POINT('',#221904);
#41358=VERTEX_POINT('',#221906);
#41359=VERTEX_POINT('',#221910);
#41360=VERTEX_POINT('',#221912);
#41361=VERTEX_POINT('',#221916);
#41362=VERTEX_POINT('',#221917);
#41363=VERTEX_POINT('',#221919);
#41364=VERTEX_POINT('',#221921);
#41365=VERTEX_POINT('',#221925);
#41366=VERTEX_POINT('',#221926);
#41367=VERTEX_POINT('',#221928);
#41368=VERTEX_POINT('',#221930);
#41369=VERTEX_POINT('',#221932);
#41370=VERTEX_POINT('',#221934);
#41371=VERTEX_POINT('',#221938);
#41372=VERTEX_POINT('',#221940);
#41373=VERTEX_POINT('',#221956);
#41374=VERTEX_POINT('',#221957);
#41375=VERTEX_POINT('',#221959);
#41376=VERTEX_POINT('',#221961);
#41377=VERTEX_POINT('',#221963);
#41378=VERTEX_POINT('',#221965);
#41379=VERTEX_POINT('',#221969);
#41380=VERTEX_POINT('',#221971);
#41381=VERTEX_POINT('',#221975);
#41382=VERTEX_POINT('',#221976);
#41383=VERTEX_POINT('',#221978);
#41384=VERTEX_POINT('',#221980);
#41385=VERTEX_POINT('',#221984);
#41386=VERTEX_POINT('',#221985);
#41387=VERTEX_POINT('',#221987);
#41388=VERTEX_POINT('',#221989);
#41389=VERTEX_POINT('',#221991);
#41390=VERTEX_POINT('',#221993);
#41391=VERTEX_POINT('',#221997);
#41392=VERTEX_POINT('',#221999);
#41393=VERTEX_POINT('',#222015);
#41394=VERTEX_POINT('',#222016);
#41395=VERTEX_POINT('',#222018);
#41396=VERTEX_POINT('',#222020);
#41397=VERTEX_POINT('',#222022);
#41398=VERTEX_POINT('',#222024);
#41399=VERTEX_POINT('',#222028);
#41400=VERTEX_POINT('',#222030);
#41401=VERTEX_POINT('',#222034);
#41402=VERTEX_POINT('',#222035);
#41403=VERTEX_POINT('',#222037);
#41404=VERTEX_POINT('',#222039);
#41405=VERTEX_POINT('',#222043);
#41406=VERTEX_POINT('',#222044);
#41407=VERTEX_POINT('',#222046);
#41408=VERTEX_POINT('',#222048);
#41409=VERTEX_POINT('',#222050);
#41410=VERTEX_POINT('',#222052);
#41411=VERTEX_POINT('',#222056);
#41412=VERTEX_POINT('',#222058);
#41413=VERTEX_POINT('',#222074);
#41414=VERTEX_POINT('',#222075);
#41415=VERTEX_POINT('',#222077);
#41416=VERTEX_POINT('',#222079);
#41417=VERTEX_POINT('',#222081);
#41418=VERTEX_POINT('',#222083);
#41419=VERTEX_POINT('',#222087);
#41420=VERTEX_POINT('',#222089);
#41421=VERTEX_POINT('',#222093);
#41422=VERTEX_POINT('',#222094);
#41423=VERTEX_POINT('',#222096);
#41424=VERTEX_POINT('',#222098);
#41425=VERTEX_POINT('',#222102);
#41426=VERTEX_POINT('',#222103);
#41427=VERTEX_POINT('',#222105);
#41428=VERTEX_POINT('',#222107);
#41429=VERTEX_POINT('',#222109);
#41430=VERTEX_POINT('',#222111);
#41431=VERTEX_POINT('',#222115);
#41432=VERTEX_POINT('',#222117);
#41433=VERTEX_POINT('',#222133);
#41434=VERTEX_POINT('',#222134);
#41435=VERTEX_POINT('',#222136);
#41436=VERTEX_POINT('',#222138);
#41437=VERTEX_POINT('',#222140);
#41438=VERTEX_POINT('',#222142);
#41439=VERTEX_POINT('',#222146);
#41440=VERTEX_POINT('',#222148);
#41441=VERTEX_POINT('',#222152);
#41442=VERTEX_POINT('',#222153);
#41443=VERTEX_POINT('',#222155);
#41444=VERTEX_POINT('',#222157);
#41445=VERTEX_POINT('',#222161);
#41446=VERTEX_POINT('',#222162);
#41447=VERTEX_POINT('',#222164);
#41448=VERTEX_POINT('',#222166);
#41449=VERTEX_POINT('',#222168);
#41450=VERTEX_POINT('',#222170);
#41451=VERTEX_POINT('',#222174);
#41452=VERTEX_POINT('',#222176);
#41453=VERTEX_POINT('',#222192);
#41454=VERTEX_POINT('',#222193);
#41455=VERTEX_POINT('',#222195);
#41456=VERTEX_POINT('',#222197);
#41457=VERTEX_POINT('',#222199);
#41458=VERTEX_POINT('',#222201);
#41459=VERTEX_POINT('',#222205);
#41460=VERTEX_POINT('',#222207);
#41461=VERTEX_POINT('',#222211);
#41462=VERTEX_POINT('',#222212);
#41463=VERTEX_POINT('',#222214);
#41464=VERTEX_POINT('',#222216);
#41465=VERTEX_POINT('',#222220);
#41466=VERTEX_POINT('',#222221);
#41467=VERTEX_POINT('',#222223);
#41468=VERTEX_POINT('',#222225);
#41469=VERTEX_POINT('',#222227);
#41470=VERTEX_POINT('',#222229);
#41471=VERTEX_POINT('',#222233);
#41472=VERTEX_POINT('',#222235);
#41473=VERTEX_POINT('',#222251);
#41474=VERTEX_POINT('',#222252);
#41475=VERTEX_POINT('',#222254);
#41476=VERTEX_POINT('',#222256);
#41477=VERTEX_POINT('',#222258);
#41478=VERTEX_POINT('',#222260);
#41479=VERTEX_POINT('',#222264);
#41480=VERTEX_POINT('',#222266);
#41481=VERTEX_POINT('',#222270);
#41482=VERTEX_POINT('',#222271);
#41483=VERTEX_POINT('',#222273);
#41484=VERTEX_POINT('',#222275);
#41485=VERTEX_POINT('',#222279);
#41486=VERTEX_POINT('',#222280);
#41487=VERTEX_POINT('',#222282);
#41488=VERTEX_POINT('',#222284);
#41489=VERTEX_POINT('',#222286);
#41490=VERTEX_POINT('',#222288);
#41491=VERTEX_POINT('',#222292);
#41492=VERTEX_POINT('',#222294);
#41493=VERTEX_POINT('',#222310);
#41494=VERTEX_POINT('',#222311);
#41495=VERTEX_POINT('',#222313);
#41496=VERTEX_POINT('',#222315);
#41497=VERTEX_POINT('',#222317);
#41498=VERTEX_POINT('',#222319);
#41499=VERTEX_POINT('',#222323);
#41500=VERTEX_POINT('',#222325);
#41501=VERTEX_POINT('',#222329);
#41502=VERTEX_POINT('',#222330);
#41503=VERTEX_POINT('',#222332);
#41504=VERTEX_POINT('',#222334);
#41505=VERTEX_POINT('',#222338);
#41506=VERTEX_POINT('',#222339);
#41507=VERTEX_POINT('',#222341);
#41508=VERTEX_POINT('',#222343);
#41509=VERTEX_POINT('',#222345);
#41510=VERTEX_POINT('',#222347);
#41511=VERTEX_POINT('',#222351);
#41512=VERTEX_POINT('',#222353);
#41513=VERTEX_POINT('',#222369);
#41514=VERTEX_POINT('',#222370);
#41515=VERTEX_POINT('',#222372);
#41516=VERTEX_POINT('',#222374);
#41517=VERTEX_POINT('',#222376);
#41518=VERTEX_POINT('',#222378);
#41519=VERTEX_POINT('',#222382);
#41520=VERTEX_POINT('',#222384);
#41521=VERTEX_POINT('',#222388);
#41522=VERTEX_POINT('',#222389);
#41523=VERTEX_POINT('',#222391);
#41524=VERTEX_POINT('',#222393);
#41525=VERTEX_POINT('',#222397);
#41526=VERTEX_POINT('',#222398);
#41527=VERTEX_POINT('',#222400);
#41528=VERTEX_POINT('',#222402);
#41529=VERTEX_POINT('',#222404);
#41530=VERTEX_POINT('',#222406);
#41531=VERTEX_POINT('',#222410);
#41532=VERTEX_POINT('',#222412);
#41533=VERTEX_POINT('',#222428);
#41534=VERTEX_POINT('',#222429);
#41535=VERTEX_POINT('',#222431);
#41536=VERTEX_POINT('',#222433);
#41537=VERTEX_POINT('',#222435);
#41538=VERTEX_POINT('',#222437);
#41539=VERTEX_POINT('',#222441);
#41540=VERTEX_POINT('',#222443);
#41541=VERTEX_POINT('',#222447);
#41542=VERTEX_POINT('',#222448);
#41543=VERTEX_POINT('',#222450);
#41544=VERTEX_POINT('',#222452);
#41545=VERTEX_POINT('',#222456);
#41546=VERTEX_POINT('',#222457);
#41547=VERTEX_POINT('',#222459);
#41548=VERTEX_POINT('',#222461);
#41549=VERTEX_POINT('',#222463);
#41550=VERTEX_POINT('',#222465);
#41551=VERTEX_POINT('',#222469);
#41552=VERTEX_POINT('',#222471);
#41553=VERTEX_POINT('',#222487);
#41554=VERTEX_POINT('',#222488);
#41555=VERTEX_POINT('',#222490);
#41556=VERTEX_POINT('',#222492);
#41557=VERTEX_POINT('',#222494);
#41558=VERTEX_POINT('',#222496);
#41559=VERTEX_POINT('',#222500);
#41560=VERTEX_POINT('',#222502);
#41561=VERTEX_POINT('',#222506);
#41562=VERTEX_POINT('',#222507);
#41563=VERTEX_POINT('',#222509);
#41564=VERTEX_POINT('',#222511);
#41565=VERTEX_POINT('',#222515);
#41566=VERTEX_POINT('',#222516);
#41567=VERTEX_POINT('',#222518);
#41568=VERTEX_POINT('',#222520);
#41569=VERTEX_POINT('',#222522);
#41570=VERTEX_POINT('',#222524);
#41571=VERTEX_POINT('',#222528);
#41572=VERTEX_POINT('',#222530);
#41573=VERTEX_POINT('',#222546);
#41574=VERTEX_POINT('',#222547);
#41575=VERTEX_POINT('',#222549);
#41576=VERTEX_POINT('',#222551);
#41577=VERTEX_POINT('',#222553);
#41578=VERTEX_POINT('',#222555);
#41579=VERTEX_POINT('',#222559);
#41580=VERTEX_POINT('',#222561);
#41581=VERTEX_POINT('',#222565);
#41582=VERTEX_POINT('',#222566);
#41583=VERTEX_POINT('',#222568);
#41584=VERTEX_POINT('',#222570);
#41585=VERTEX_POINT('',#222574);
#41586=VERTEX_POINT('',#222575);
#41587=VERTEX_POINT('',#222577);
#41588=VERTEX_POINT('',#222579);
#41589=VERTEX_POINT('',#222581);
#41590=VERTEX_POINT('',#222583);
#41591=VERTEX_POINT('',#222587);
#41592=VERTEX_POINT('',#222589);
#41593=VERTEX_POINT('',#222605);
#41594=VERTEX_POINT('',#222606);
#41595=VERTEX_POINT('',#222608);
#41596=VERTEX_POINT('',#222610);
#41597=VERTEX_POINT('',#222612);
#41598=VERTEX_POINT('',#222614);
#41599=VERTEX_POINT('',#222618);
#41600=VERTEX_POINT('',#222620);
#41601=VERTEX_POINT('',#222624);
#41602=VERTEX_POINT('',#222625);
#41603=VERTEX_POINT('',#222627);
#41604=VERTEX_POINT('',#222629);
#41605=VERTEX_POINT('',#222633);
#41606=VERTEX_POINT('',#222634);
#41607=VERTEX_POINT('',#222636);
#41608=VERTEX_POINT('',#222638);
#41609=VERTEX_POINT('',#222640);
#41610=VERTEX_POINT('',#222642);
#41611=VERTEX_POINT('',#222646);
#41612=VERTEX_POINT('',#222648);
#41613=VERTEX_POINT('',#222664);
#41614=VERTEX_POINT('',#222665);
#41615=VERTEX_POINT('',#222667);
#41616=VERTEX_POINT('',#222669);
#41617=VERTEX_POINT('',#222671);
#41618=VERTEX_POINT('',#222673);
#41619=VERTEX_POINT('',#222677);
#41620=VERTEX_POINT('',#222679);
#41621=VERTEX_POINT('',#222683);
#41622=VERTEX_POINT('',#222684);
#41623=VERTEX_POINT('',#222686);
#41624=VERTEX_POINT('',#222688);
#41625=VERTEX_POINT('',#222692);
#41626=VERTEX_POINT('',#222693);
#41627=VERTEX_POINT('',#222695);
#41628=VERTEX_POINT('',#222697);
#41629=VERTEX_POINT('',#222699);
#41630=VERTEX_POINT('',#222701);
#41631=VERTEX_POINT('',#222705);
#41632=VERTEX_POINT('',#222707);
#41633=VERTEX_POINT('',#222723);
#41634=VERTEX_POINT('',#222724);
#41635=VERTEX_POINT('',#222726);
#41636=VERTEX_POINT('',#222728);
#41637=VERTEX_POINT('',#222730);
#41638=VERTEX_POINT('',#222732);
#41639=VERTEX_POINT('',#222736);
#41640=VERTEX_POINT('',#222738);
#41641=VERTEX_POINT('',#222742);
#41642=VERTEX_POINT('',#222743);
#41643=VERTEX_POINT('',#222745);
#41644=VERTEX_POINT('',#222747);
#41645=VERTEX_POINT('',#222751);
#41646=VERTEX_POINT('',#222752);
#41647=VERTEX_POINT('',#222754);
#41648=VERTEX_POINT('',#222756);
#41649=VERTEX_POINT('',#222758);
#41650=VERTEX_POINT('',#222760);
#41651=VERTEX_POINT('',#222764);
#41652=VERTEX_POINT('',#222766);
#41653=VERTEX_POINT('',#222782);
#41654=VERTEX_POINT('',#222783);
#41655=VERTEX_POINT('',#222785);
#41656=VERTEX_POINT('',#222787);
#41657=VERTEX_POINT('',#222789);
#41658=VERTEX_POINT('',#222791);
#41659=VERTEX_POINT('',#222795);
#41660=VERTEX_POINT('',#222797);
#41661=VERTEX_POINT('',#222801);
#41662=VERTEX_POINT('',#222802);
#41663=VERTEX_POINT('',#222804);
#41664=VERTEX_POINT('',#222806);
#41665=VERTEX_POINT('',#222810);
#41666=VERTEX_POINT('',#222811);
#41667=VERTEX_POINT('',#222813);
#41668=VERTEX_POINT('',#222815);
#41669=VERTEX_POINT('',#222817);
#41670=VERTEX_POINT('',#222819);
#41671=VERTEX_POINT('',#222823);
#41672=VERTEX_POINT('',#222825);
#41673=VERTEX_POINT('',#222841);
#41674=VERTEX_POINT('',#222842);
#41675=VERTEX_POINT('',#222844);
#41676=VERTEX_POINT('',#222846);
#41677=VERTEX_POINT('',#222848);
#41678=VERTEX_POINT('',#222850);
#41679=VERTEX_POINT('',#222854);
#41680=VERTEX_POINT('',#222856);
#41681=VERTEX_POINT('',#222860);
#41682=VERTEX_POINT('',#222861);
#41683=VERTEX_POINT('',#222863);
#41684=VERTEX_POINT('',#222865);
#41685=VERTEX_POINT('',#222869);
#41686=VERTEX_POINT('',#222870);
#41687=VERTEX_POINT('',#222872);
#41688=VERTEX_POINT('',#222874);
#41689=VERTEX_POINT('',#222876);
#41690=VERTEX_POINT('',#222878);
#41691=VERTEX_POINT('',#222882);
#41692=VERTEX_POINT('',#222884);
#41693=VERTEX_POINT('',#222900);
#41694=VERTEX_POINT('',#222901);
#41695=VERTEX_POINT('',#222903);
#41696=VERTEX_POINT('',#222905);
#41697=VERTEX_POINT('',#222907);
#41698=VERTEX_POINT('',#222909);
#41699=VERTEX_POINT('',#222913);
#41700=VERTEX_POINT('',#222915);
#41701=VERTEX_POINT('',#222919);
#41702=VERTEX_POINT('',#222920);
#41703=VERTEX_POINT('',#222922);
#41704=VERTEX_POINT('',#222924);
#41705=VERTEX_POINT('',#222928);
#41706=VERTEX_POINT('',#222929);
#41707=VERTEX_POINT('',#222931);
#41708=VERTEX_POINT('',#222933);
#41709=VERTEX_POINT('',#222935);
#41710=VERTEX_POINT('',#222937);
#41711=VERTEX_POINT('',#222941);
#41712=VERTEX_POINT('',#222943);
#41713=VERTEX_POINT('',#222959);
#41714=VERTEX_POINT('',#222960);
#41715=VERTEX_POINT('',#222962);
#41716=VERTEX_POINT('',#222964);
#41717=VERTEX_POINT('',#222966);
#41718=VERTEX_POINT('',#222968);
#41719=VERTEX_POINT('',#222972);
#41720=VERTEX_POINT('',#222974);
#41721=VERTEX_POINT('',#222978);
#41722=VERTEX_POINT('',#222979);
#41723=VERTEX_POINT('',#222981);
#41724=VERTEX_POINT('',#222983);
#41725=VERTEX_POINT('',#222987);
#41726=VERTEX_POINT('',#222988);
#41727=VERTEX_POINT('',#222990);
#41728=VERTEX_POINT('',#222992);
#41729=VERTEX_POINT('',#222994);
#41730=VERTEX_POINT('',#222996);
#41731=VERTEX_POINT('',#223000);
#41732=VERTEX_POINT('',#223002);
#41733=VERTEX_POINT('',#223018);
#41734=VERTEX_POINT('',#223019);
#41735=VERTEX_POINT('',#223021);
#41736=VERTEX_POINT('',#223023);
#41737=VERTEX_POINT('',#223025);
#41738=VERTEX_POINT('',#223027);
#41739=VERTEX_POINT('',#223031);
#41740=VERTEX_POINT('',#223033);
#41741=VERTEX_POINT('',#223037);
#41742=VERTEX_POINT('',#223038);
#41743=VERTEX_POINT('',#223040);
#41744=VERTEX_POINT('',#223042);
#41745=VERTEX_POINT('',#223046);
#41746=VERTEX_POINT('',#223047);
#41747=VERTEX_POINT('',#223049);
#41748=VERTEX_POINT('',#223051);
#41749=VERTEX_POINT('',#223053);
#41750=VERTEX_POINT('',#223055);
#41751=VERTEX_POINT('',#223059);
#41752=VERTEX_POINT('',#223061);
#41753=VERTEX_POINT('',#223077);
#41754=VERTEX_POINT('',#223078);
#41755=VERTEX_POINT('',#223080);
#41756=VERTEX_POINT('',#223082);
#41757=VERTEX_POINT('',#223084);
#41758=VERTEX_POINT('',#223086);
#41759=VERTEX_POINT('',#223090);
#41760=VERTEX_POINT('',#223092);
#41761=VERTEX_POINT('',#223096);
#41762=VERTEX_POINT('',#223097);
#41763=VERTEX_POINT('',#223099);
#41764=VERTEX_POINT('',#223101);
#41765=VERTEX_POINT('',#223105);
#41766=VERTEX_POINT('',#223106);
#41767=VERTEX_POINT('',#223108);
#41768=VERTEX_POINT('',#223110);
#41769=VERTEX_POINT('',#223112);
#41770=VERTEX_POINT('',#223114);
#41771=VERTEX_POINT('',#223118);
#41772=VERTEX_POINT('',#223120);
#41773=VERTEX_POINT('',#223136);
#41774=VERTEX_POINT('',#223137);
#41775=VERTEX_POINT('',#223139);
#41776=VERTEX_POINT('',#223141);
#41777=VERTEX_POINT('',#223143);
#41778=VERTEX_POINT('',#223145);
#41779=VERTEX_POINT('',#223149);
#41780=VERTEX_POINT('',#223151);
#41781=VERTEX_POINT('',#223155);
#41782=VERTEX_POINT('',#223156);
#41783=VERTEX_POINT('',#223158);
#41784=VERTEX_POINT('',#223160);
#41785=VERTEX_POINT('',#223164);
#41786=VERTEX_POINT('',#223165);
#41787=VERTEX_POINT('',#223167);
#41788=VERTEX_POINT('',#223169);
#41789=VERTEX_POINT('',#223171);
#41790=VERTEX_POINT('',#223173);
#41791=VERTEX_POINT('',#223177);
#41792=VERTEX_POINT('',#223179);
#41793=VERTEX_POINT('',#223195);
#41794=VERTEX_POINT('',#223196);
#41795=VERTEX_POINT('',#223198);
#41796=VERTEX_POINT('',#223200);
#41797=VERTEX_POINT('',#223202);
#41798=VERTEX_POINT('',#223204);
#41799=VERTEX_POINT('',#223208);
#41800=VERTEX_POINT('',#223210);
#41801=VERTEX_POINT('',#223214);
#41802=VERTEX_POINT('',#223215);
#41803=VERTEX_POINT('',#223217);
#41804=VERTEX_POINT('',#223219);
#41805=VERTEX_POINT('',#223223);
#41806=VERTEX_POINT('',#223224);
#41807=VERTEX_POINT('',#223226);
#41808=VERTEX_POINT('',#223228);
#41809=VERTEX_POINT('',#223230);
#41810=VERTEX_POINT('',#223232);
#41811=VERTEX_POINT('',#223236);
#41812=VERTEX_POINT('',#223238);
#41813=VERTEX_POINT('',#223254);
#41814=VERTEX_POINT('',#223255);
#41815=VERTEX_POINT('',#223257);
#41816=VERTEX_POINT('',#223259);
#41817=VERTEX_POINT('',#223261);
#41818=VERTEX_POINT('',#223263);
#41819=VERTEX_POINT('',#223267);
#41820=VERTEX_POINT('',#223269);
#41821=VERTEX_POINT('',#223273);
#41822=VERTEX_POINT('',#223274);
#41823=VERTEX_POINT('',#223276);
#41824=VERTEX_POINT('',#223278);
#41825=VERTEX_POINT('',#223282);
#41826=VERTEX_POINT('',#223283);
#41827=VERTEX_POINT('',#223285);
#41828=VERTEX_POINT('',#223287);
#41829=VERTEX_POINT('',#223289);
#41830=VERTEX_POINT('',#223291);
#41831=VERTEX_POINT('',#223295);
#41832=VERTEX_POINT('',#223297);
#41833=VERTEX_POINT('',#223313);
#41834=VERTEX_POINT('',#223314);
#41835=VERTEX_POINT('',#223316);
#41836=VERTEX_POINT('',#223318);
#41837=VERTEX_POINT('',#223320);
#41838=VERTEX_POINT('',#223322);
#41839=VERTEX_POINT('',#223326);
#41840=VERTEX_POINT('',#223328);
#41841=VERTEX_POINT('',#223332);
#41842=VERTEX_POINT('',#223333);
#41843=VERTEX_POINT('',#223335);
#41844=VERTEX_POINT('',#223337);
#41845=VERTEX_POINT('',#223341);
#41846=VERTEX_POINT('',#223342);
#41847=VERTEX_POINT('',#223344);
#41848=VERTEX_POINT('',#223346);
#41849=VERTEX_POINT('',#223348);
#41850=VERTEX_POINT('',#223350);
#41851=VERTEX_POINT('',#223354);
#41852=VERTEX_POINT('',#223356);
#41853=VERTEX_POINT('',#223372);
#41854=VERTEX_POINT('',#223373);
#41855=VERTEX_POINT('',#223375);
#41856=VERTEX_POINT('',#223377);
#41857=VERTEX_POINT('',#223379);
#41858=VERTEX_POINT('',#223381);
#41859=VERTEX_POINT('',#223385);
#41860=VERTEX_POINT('',#223387);
#41861=VERTEX_POINT('',#223391);
#41862=VERTEX_POINT('',#223392);
#41863=VERTEX_POINT('',#223394);
#41864=VERTEX_POINT('',#223396);
#41865=VERTEX_POINT('',#223400);
#41866=VERTEX_POINT('',#223401);
#41867=VERTEX_POINT('',#223403);
#41868=VERTEX_POINT('',#223405);
#41869=VERTEX_POINT('',#223407);
#41870=VERTEX_POINT('',#223409);
#41871=VERTEX_POINT('',#223413);
#41872=VERTEX_POINT('',#223415);
#41873=VERTEX_POINT('',#223431);
#41874=VERTEX_POINT('',#223432);
#41875=VERTEX_POINT('',#223434);
#41876=VERTEX_POINT('',#223436);
#41877=VERTEX_POINT('',#223438);
#41878=VERTEX_POINT('',#223440);
#41879=VERTEX_POINT('',#223444);
#41880=VERTEX_POINT('',#223446);
#41881=VERTEX_POINT('',#223450);
#41882=VERTEX_POINT('',#223451);
#41883=VERTEX_POINT('',#223453);
#41884=VERTEX_POINT('',#223455);
#41885=VERTEX_POINT('',#223459);
#41886=VERTEX_POINT('',#223460);
#41887=VERTEX_POINT('',#223462);
#41888=VERTEX_POINT('',#223464);
#41889=VERTEX_POINT('',#223466);
#41890=VERTEX_POINT('',#223468);
#41891=VERTEX_POINT('',#223472);
#41892=VERTEX_POINT('',#223474);
#41893=VERTEX_POINT('',#223490);
#41894=VERTEX_POINT('',#223491);
#41895=VERTEX_POINT('',#223493);
#41896=VERTEX_POINT('',#223495);
#41897=VERTEX_POINT('',#223497);
#41898=VERTEX_POINT('',#223499);
#41899=VERTEX_POINT('',#223503);
#41900=VERTEX_POINT('',#223505);
#41901=VERTEX_POINT('',#223509);
#41902=VERTEX_POINT('',#223510);
#41903=VERTEX_POINT('',#223512);
#41904=VERTEX_POINT('',#223514);
#41905=VERTEX_POINT('',#223518);
#41906=VERTEX_POINT('',#223519);
#41907=VERTEX_POINT('',#223521);
#41908=VERTEX_POINT('',#223523);
#41909=VERTEX_POINT('',#223525);
#41910=VERTEX_POINT('',#223527);
#41911=VERTEX_POINT('',#223531);
#41912=VERTEX_POINT('',#223533);
#41913=VERTEX_POINT('',#223549);
#41914=VERTEX_POINT('',#223550);
#41915=VERTEX_POINT('',#223552);
#41916=VERTEX_POINT('',#223554);
#41917=VERTEX_POINT('',#223556);
#41918=VERTEX_POINT('',#223558);
#41919=VERTEX_POINT('',#223562);
#41920=VERTEX_POINT('',#223564);
#41921=VERTEX_POINT('',#223568);
#41922=VERTEX_POINT('',#223569);
#41923=VERTEX_POINT('',#223571);
#41924=VERTEX_POINT('',#223573);
#41925=VERTEX_POINT('',#223577);
#41926=VERTEX_POINT('',#223578);
#41927=VERTEX_POINT('',#223580);
#41928=VERTEX_POINT('',#223582);
#41929=VERTEX_POINT('',#223584);
#41930=VERTEX_POINT('',#223586);
#41931=VERTEX_POINT('',#223590);
#41932=VERTEX_POINT('',#223592);
#41933=VERTEX_POINT('',#223608);
#41934=VERTEX_POINT('',#223609);
#41935=VERTEX_POINT('',#223611);
#41936=VERTEX_POINT('',#223613);
#41937=VERTEX_POINT('',#223615);
#41938=VERTEX_POINT('',#223617);
#41939=VERTEX_POINT('',#223621);
#41940=VERTEX_POINT('',#223623);
#41941=VERTEX_POINT('',#223627);
#41942=VERTEX_POINT('',#223628);
#41943=VERTEX_POINT('',#223630);
#41944=VERTEX_POINT('',#223632);
#41945=VERTEX_POINT('',#223636);
#41946=VERTEX_POINT('',#223637);
#41947=VERTEX_POINT('',#223639);
#41948=VERTEX_POINT('',#223641);
#41949=VERTEX_POINT('',#223643);
#41950=VERTEX_POINT('',#223645);
#41951=VERTEX_POINT('',#223649);
#41952=VERTEX_POINT('',#223651);
#41953=VERTEX_POINT('',#223667);
#41954=VERTEX_POINT('',#223668);
#41955=VERTEX_POINT('',#223670);
#41956=VERTEX_POINT('',#223672);
#41957=VERTEX_POINT('',#223674);
#41958=VERTEX_POINT('',#223676);
#41959=VERTEX_POINT('',#223680);
#41960=VERTEX_POINT('',#223682);
#41961=VERTEX_POINT('',#223686);
#41962=VERTEX_POINT('',#223687);
#41963=VERTEX_POINT('',#223689);
#41964=VERTEX_POINT('',#223691);
#41965=VERTEX_POINT('',#223695);
#41966=VERTEX_POINT('',#223696);
#41967=VERTEX_POINT('',#223698);
#41968=VERTEX_POINT('',#223700);
#41969=VERTEX_POINT('',#223702);
#41970=VERTEX_POINT('',#223704);
#41971=VERTEX_POINT('',#223708);
#41972=VERTEX_POINT('',#223710);
#41973=VERTEX_POINT('',#223726);
#41974=VERTEX_POINT('',#223727);
#41975=VERTEX_POINT('',#223729);
#41976=VERTEX_POINT('',#223731);
#41977=VERTEX_POINT('',#223733);
#41978=VERTEX_POINT('',#223735);
#41979=VERTEX_POINT('',#223739);
#41980=VERTEX_POINT('',#223741);
#41981=VERTEX_POINT('',#223745);
#41982=VERTEX_POINT('',#223746);
#41983=VERTEX_POINT('',#223748);
#41984=VERTEX_POINT('',#223750);
#41985=VERTEX_POINT('',#223754);
#41986=VERTEX_POINT('',#223755);
#41987=VERTEX_POINT('',#223757);
#41988=VERTEX_POINT('',#223759);
#41989=VERTEX_POINT('',#223761);
#41990=VERTEX_POINT('',#223763);
#41991=VERTEX_POINT('',#223767);
#41992=VERTEX_POINT('',#223769);
#41993=VERTEX_POINT('',#223785);
#41994=VERTEX_POINT('',#223786);
#41995=VERTEX_POINT('',#223788);
#41996=VERTEX_POINT('',#223790);
#41997=VERTEX_POINT('',#223792);
#41998=VERTEX_POINT('',#223794);
#41999=VERTEX_POINT('',#223798);
#42000=VERTEX_POINT('',#223800);
#42001=VERTEX_POINT('',#223804);
#42002=VERTEX_POINT('',#223805);
#42003=VERTEX_POINT('',#223807);
#42004=VERTEX_POINT('',#223809);
#42005=VERTEX_POINT('',#223813);
#42006=VERTEX_POINT('',#223814);
#42007=VERTEX_POINT('',#223816);
#42008=VERTEX_POINT('',#223818);
#42009=VERTEX_POINT('',#223820);
#42010=VERTEX_POINT('',#223822);
#42011=VERTEX_POINT('',#223826);
#42012=VERTEX_POINT('',#223828);
#42013=VERTEX_POINT('',#223844);
#42014=VERTEX_POINT('',#223845);
#42015=VERTEX_POINT('',#223847);
#42016=VERTEX_POINT('',#223849);
#42017=VERTEX_POINT('',#223851);
#42018=VERTEX_POINT('',#223853);
#42019=VERTEX_POINT('',#223857);
#42020=VERTEX_POINT('',#223859);
#42021=VERTEX_POINT('',#223863);
#42022=VERTEX_POINT('',#223864);
#42023=VERTEX_POINT('',#223866);
#42024=VERTEX_POINT('',#223868);
#42025=VERTEX_POINT('',#223872);
#42026=VERTEX_POINT('',#223873);
#42027=VERTEX_POINT('',#223875);
#42028=VERTEX_POINT('',#223877);
#42029=VERTEX_POINT('',#223879);
#42030=VERTEX_POINT('',#223881);
#42031=VERTEX_POINT('',#223885);
#42032=VERTEX_POINT('',#223887);
#42033=VERTEX_POINT('',#223903);
#42034=VERTEX_POINT('',#223904);
#42035=VERTEX_POINT('',#223906);
#42036=VERTEX_POINT('',#223908);
#42037=VERTEX_POINT('',#223910);
#42038=VERTEX_POINT('',#223912);
#42039=VERTEX_POINT('',#223916);
#42040=VERTEX_POINT('',#223918);
#42041=VERTEX_POINT('',#223922);
#42042=VERTEX_POINT('',#223923);
#42043=VERTEX_POINT('',#223925);
#42044=VERTEX_POINT('',#223927);
#42045=VERTEX_POINT('',#223931);
#42046=VERTEX_POINT('',#223932);
#42047=VERTEX_POINT('',#223934);
#42048=VERTEX_POINT('',#223936);
#42049=VERTEX_POINT('',#223938);
#42050=VERTEX_POINT('',#223940);
#42051=VERTEX_POINT('',#223944);
#42052=VERTEX_POINT('',#223946);
#42053=VERTEX_POINT('',#223962);
#42054=VERTEX_POINT('',#223963);
#42055=VERTEX_POINT('',#223965);
#42056=VERTEX_POINT('',#223967);
#42057=VERTEX_POINT('',#223969);
#42058=VERTEX_POINT('',#223971);
#42059=VERTEX_POINT('',#223975);
#42060=VERTEX_POINT('',#223977);
#42061=VERTEX_POINT('',#223981);
#42062=VERTEX_POINT('',#223982);
#42063=VERTEX_POINT('',#223984);
#42064=VERTEX_POINT('',#223986);
#42065=VERTEX_POINT('',#223990);
#42066=VERTEX_POINT('',#223991);
#42067=VERTEX_POINT('',#223993);
#42068=VERTEX_POINT('',#223995);
#42069=VERTEX_POINT('',#223997);
#42070=VERTEX_POINT('',#223999);
#42071=VERTEX_POINT('',#224003);
#42072=VERTEX_POINT('',#224005);
#42073=VERTEX_POINT('',#224021);
#42074=VERTEX_POINT('',#224022);
#42075=VERTEX_POINT('',#224024);
#42076=VERTEX_POINT('',#224026);
#42077=VERTEX_POINT('',#224028);
#42078=VERTEX_POINT('',#224030);
#42079=VERTEX_POINT('',#224034);
#42080=VERTEX_POINT('',#224036);
#42081=VERTEX_POINT('',#224040);
#42082=VERTEX_POINT('',#224041);
#42083=VERTEX_POINT('',#224043);
#42084=VERTEX_POINT('',#224045);
#42085=VERTEX_POINT('',#224049);
#42086=VERTEX_POINT('',#224050);
#42087=VERTEX_POINT('',#224052);
#42088=VERTEX_POINT('',#224054);
#42089=VERTEX_POINT('',#224056);
#42090=VERTEX_POINT('',#224058);
#42091=VERTEX_POINT('',#224062);
#42092=VERTEX_POINT('',#224064);
#42093=VERTEX_POINT('',#224080);
#42094=VERTEX_POINT('',#224081);
#42095=VERTEX_POINT('',#224083);
#42096=VERTEX_POINT('',#224085);
#42097=VERTEX_POINT('',#224087);
#42098=VERTEX_POINT('',#224089);
#42099=VERTEX_POINT('',#224093);
#42100=VERTEX_POINT('',#224095);
#42101=VERTEX_POINT('',#224099);
#42102=VERTEX_POINT('',#224100);
#42103=VERTEX_POINT('',#224102);
#42104=VERTEX_POINT('',#224104);
#42105=VERTEX_POINT('',#224108);
#42106=VERTEX_POINT('',#224109);
#42107=VERTEX_POINT('',#224111);
#42108=VERTEX_POINT('',#224113);
#42109=VERTEX_POINT('',#224115);
#42110=VERTEX_POINT('',#224117);
#42111=VERTEX_POINT('',#224121);
#42112=VERTEX_POINT('',#224123);
#42113=VERTEX_POINT('',#224139);
#42114=VERTEX_POINT('',#224140);
#42115=VERTEX_POINT('',#224142);
#42116=VERTEX_POINT('',#224144);
#42117=VERTEX_POINT('',#224146);
#42118=VERTEX_POINT('',#224148);
#42119=VERTEX_POINT('',#224152);
#42120=VERTEX_POINT('',#224154);
#42121=VERTEX_POINT('',#224158);
#42122=VERTEX_POINT('',#224159);
#42123=VERTEX_POINT('',#224161);
#42124=VERTEX_POINT('',#224163);
#42125=VERTEX_POINT('',#224167);
#42126=VERTEX_POINT('',#224168);
#42127=VERTEX_POINT('',#224170);
#42128=VERTEX_POINT('',#224172);
#42129=VERTEX_POINT('',#224174);
#42130=VERTEX_POINT('',#224176);
#42131=VERTEX_POINT('',#224180);
#42132=VERTEX_POINT('',#224182);
#42133=VERTEX_POINT('',#224198);
#42134=VERTEX_POINT('',#224199);
#42135=VERTEX_POINT('',#224201);
#42136=VERTEX_POINT('',#224203);
#42137=VERTEX_POINT('',#224205);
#42138=VERTEX_POINT('',#224207);
#42139=VERTEX_POINT('',#224211);
#42140=VERTEX_POINT('',#224213);
#42141=VERTEX_POINT('',#224217);
#42142=VERTEX_POINT('',#224218);
#42143=VERTEX_POINT('',#224220);
#42144=VERTEX_POINT('',#224222);
#42145=VERTEX_POINT('',#224226);
#42146=VERTEX_POINT('',#224227);
#42147=VERTEX_POINT('',#224229);
#42148=VERTEX_POINT('',#224231);
#42149=VERTEX_POINT('',#224233);
#42150=VERTEX_POINT('',#224235);
#42151=VERTEX_POINT('',#224239);
#42152=VERTEX_POINT('',#224241);
#42153=VERTEX_POINT('',#224257);
#42154=VERTEX_POINT('',#224258);
#42155=VERTEX_POINT('',#224260);
#42156=VERTEX_POINT('',#224262);
#42157=VERTEX_POINT('',#224264);
#42158=VERTEX_POINT('',#224266);
#42159=VERTEX_POINT('',#224270);
#42160=VERTEX_POINT('',#224272);
#42161=VERTEX_POINT('',#224276);
#42162=VERTEX_POINT('',#224277);
#42163=VERTEX_POINT('',#224279);
#42164=VERTEX_POINT('',#224281);
#42165=VERTEX_POINT('',#224285);
#42166=VERTEX_POINT('',#224286);
#42167=VERTEX_POINT('',#224288);
#42168=VERTEX_POINT('',#224290);
#42169=VERTEX_POINT('',#224292);
#42170=VERTEX_POINT('',#224294);
#42171=VERTEX_POINT('',#224298);
#42172=VERTEX_POINT('',#224300);
#42173=VERTEX_POINT('',#224316);
#42174=VERTEX_POINT('',#224317);
#42175=VERTEX_POINT('',#224319);
#42176=VERTEX_POINT('',#224321);
#42177=VERTEX_POINT('',#224323);
#42178=VERTEX_POINT('',#224325);
#42179=VERTEX_POINT('',#224329);
#42180=VERTEX_POINT('',#224331);
#42181=VERTEX_POINT('',#224335);
#42182=VERTEX_POINT('',#224336);
#42183=VERTEX_POINT('',#224338);
#42184=VERTEX_POINT('',#224340);
#42185=VERTEX_POINT('',#224344);
#42186=VERTEX_POINT('',#224345);
#42187=VERTEX_POINT('',#224347);
#42188=VERTEX_POINT('',#224349);
#42189=VERTEX_POINT('',#224351);
#42190=VERTEX_POINT('',#224353);
#42191=VERTEX_POINT('',#224357);
#42192=VERTEX_POINT('',#224359);
#42193=VERTEX_POINT('',#224375);
#42194=VERTEX_POINT('',#224376);
#42195=VERTEX_POINT('',#224378);
#42196=VERTEX_POINT('',#224380);
#42197=VERTEX_POINT('',#224382);
#42198=VERTEX_POINT('',#224384);
#42199=VERTEX_POINT('',#224388);
#42200=VERTEX_POINT('',#224390);
#42201=VERTEX_POINT('',#224394);
#42202=VERTEX_POINT('',#224395);
#42203=VERTEX_POINT('',#224397);
#42204=VERTEX_POINT('',#224399);
#42205=VERTEX_POINT('',#224403);
#42206=VERTEX_POINT('',#224404);
#42207=VERTEX_POINT('',#224406);
#42208=VERTEX_POINT('',#224408);
#42209=VERTEX_POINT('',#224410);
#42210=VERTEX_POINT('',#224412);
#42211=VERTEX_POINT('',#224416);
#42212=VERTEX_POINT('',#224418);
#42213=VERTEX_POINT('',#224434);
#42214=VERTEX_POINT('',#224435);
#42215=VERTEX_POINT('',#224437);
#42216=VERTEX_POINT('',#224439);
#42217=VERTEX_POINT('',#224441);
#42218=VERTEX_POINT('',#224443);
#42219=VERTEX_POINT('',#224447);
#42220=VERTEX_POINT('',#224449);
#42221=VERTEX_POINT('',#224453);
#42222=VERTEX_POINT('',#224454);
#42223=VERTEX_POINT('',#224456);
#42224=VERTEX_POINT('',#224458);
#42225=VERTEX_POINT('',#224462);
#42226=VERTEX_POINT('',#224463);
#42227=VERTEX_POINT('',#224465);
#42228=VERTEX_POINT('',#224467);
#42229=VERTEX_POINT('',#224469);
#42230=VERTEX_POINT('',#224471);
#42231=VERTEX_POINT('',#224475);
#42232=VERTEX_POINT('',#224477);
#42233=VERTEX_POINT('',#224493);
#42234=VERTEX_POINT('',#224494);
#42235=VERTEX_POINT('',#224496);
#42236=VERTEX_POINT('',#224498);
#42237=VERTEX_POINT('',#224500);
#42238=VERTEX_POINT('',#224502);
#42239=VERTEX_POINT('',#224506);
#42240=VERTEX_POINT('',#224508);
#42241=VERTEX_POINT('',#224512);
#42242=VERTEX_POINT('',#224513);
#42243=VERTEX_POINT('',#224515);
#42244=VERTEX_POINT('',#224517);
#42245=VERTEX_POINT('',#224521);
#42246=VERTEX_POINT('',#224522);
#42247=VERTEX_POINT('',#224524);
#42248=VERTEX_POINT('',#224526);
#42249=VERTEX_POINT('',#224528);
#42250=VERTEX_POINT('',#224530);
#42251=VERTEX_POINT('',#224534);
#42252=VERTEX_POINT('',#224536);
#42253=VERTEX_POINT('',#224552);
#42254=VERTEX_POINT('',#224553);
#42255=VERTEX_POINT('',#224555);
#42256=VERTEX_POINT('',#224557);
#42257=VERTEX_POINT('',#224559);
#42258=VERTEX_POINT('',#224561);
#42259=VERTEX_POINT('',#224565);
#42260=VERTEX_POINT('',#224567);
#42261=VERTEX_POINT('',#224571);
#42262=VERTEX_POINT('',#224572);
#42263=VERTEX_POINT('',#224574);
#42264=VERTEX_POINT('',#224576);
#42265=VERTEX_POINT('',#224580);
#42266=VERTEX_POINT('',#224581);
#42267=VERTEX_POINT('',#224583);
#42268=VERTEX_POINT('',#224585);
#42269=VERTEX_POINT('',#224587);
#42270=VERTEX_POINT('',#224589);
#42271=VERTEX_POINT('',#224593);
#42272=VERTEX_POINT('',#224595);
#42273=VERTEX_POINT('',#224611);
#42274=VERTEX_POINT('',#224612);
#42275=VERTEX_POINT('',#224614);
#42276=VERTEX_POINT('',#224616);
#42277=VERTEX_POINT('',#224618);
#42278=VERTEX_POINT('',#224620);
#42279=VERTEX_POINT('',#224624);
#42280=VERTEX_POINT('',#224626);
#42281=VERTEX_POINT('',#224630);
#42282=VERTEX_POINT('',#224631);
#42283=VERTEX_POINT('',#224633);
#42284=VERTEX_POINT('',#224635);
#42285=VERTEX_POINT('',#224639);
#42286=VERTEX_POINT('',#224640);
#42287=VERTEX_POINT('',#224642);
#42288=VERTEX_POINT('',#224644);
#42289=VERTEX_POINT('',#224646);
#42290=VERTEX_POINT('',#224648);
#42291=VERTEX_POINT('',#224652);
#42292=VERTEX_POINT('',#224654);
#42293=VERTEX_POINT('',#224670);
#42294=VERTEX_POINT('',#224671);
#42295=VERTEX_POINT('',#224673);
#42296=VERTEX_POINT('',#224675);
#42297=VERTEX_POINT('',#224677);
#42298=VERTEX_POINT('',#224679);
#42299=VERTEX_POINT('',#224683);
#42300=VERTEX_POINT('',#224685);
#42301=VERTEX_POINT('',#224689);
#42302=VERTEX_POINT('',#224690);
#42303=VERTEX_POINT('',#224692);
#42304=VERTEX_POINT('',#224694);
#42305=VERTEX_POINT('',#224698);
#42306=VERTEX_POINT('',#224699);
#42307=VERTEX_POINT('',#224701);
#42308=VERTEX_POINT('',#224703);
#42309=VERTEX_POINT('',#224705);
#42310=VERTEX_POINT('',#224707);
#42311=VERTEX_POINT('',#224711);
#42312=VERTEX_POINT('',#224713);
#42313=VERTEX_POINT('',#224729);
#42314=VERTEX_POINT('',#224730);
#42315=VERTEX_POINT('',#224732);
#42316=VERTEX_POINT('',#224734);
#42317=VERTEX_POINT('',#224736);
#42318=VERTEX_POINT('',#224738);
#42319=VERTEX_POINT('',#224742);
#42320=VERTEX_POINT('',#224744);
#42321=VERTEX_POINT('',#224748);
#42322=VERTEX_POINT('',#224749);
#42323=VERTEX_POINT('',#224751);
#42324=VERTEX_POINT('',#224753);
#42325=VERTEX_POINT('',#224757);
#42326=VERTEX_POINT('',#224758);
#42327=VERTEX_POINT('',#224760);
#42328=VERTEX_POINT('',#224762);
#42329=VERTEX_POINT('',#224764);
#42330=VERTEX_POINT('',#224766);
#42331=VERTEX_POINT('',#224770);
#42332=VERTEX_POINT('',#224772);
#42333=VERTEX_POINT('',#224788);
#42334=VERTEX_POINT('',#224789);
#42335=VERTEX_POINT('',#224791);
#42336=VERTEX_POINT('',#224793);
#42337=VERTEX_POINT('',#224795);
#42338=VERTEX_POINT('',#224797);
#42339=VERTEX_POINT('',#224801);
#42340=VERTEX_POINT('',#224803);
#42341=VERTEX_POINT('',#224807);
#42342=VERTEX_POINT('',#224808);
#42343=VERTEX_POINT('',#224810);
#42344=VERTEX_POINT('',#224812);
#42345=VERTEX_POINT('',#224816);
#42346=VERTEX_POINT('',#224817);
#42347=VERTEX_POINT('',#224819);
#42348=VERTEX_POINT('',#224821);
#42349=VERTEX_POINT('',#224823);
#42350=VERTEX_POINT('',#224825);
#42351=VERTEX_POINT('',#224829);
#42352=VERTEX_POINT('',#224831);
#42353=VERTEX_POINT('',#224848);
#42354=VERTEX_POINT('',#224849);
#42355=VERTEX_POINT('',#224851);
#42356=VERTEX_POINT('',#224853);
#42357=VERTEX_POINT('',#224855);
#42358=VERTEX_POINT('',#224857);
#42359=VERTEX_POINT('',#224861);
#42360=VERTEX_POINT('',#224863);
#42361=VERTEX_POINT('',#224867);
#42362=VERTEX_POINT('',#224868);
#42363=VERTEX_POINT('',#224870);
#42364=VERTEX_POINT('',#224872);
#42365=VERTEX_POINT('',#224876);
#42366=VERTEX_POINT('',#224877);
#42367=VERTEX_POINT('',#224879);
#42368=VERTEX_POINT('',#224881);
#42369=VERTEX_POINT('',#224883);
#42370=VERTEX_POINT('',#224885);
#42371=VERTEX_POINT('',#224889);
#42372=VERTEX_POINT('',#224891);
#42373=VERTEX_POINT('',#224909);
#42374=VERTEX_POINT('',#224910);
#42375=VERTEX_POINT('',#224912);
#42376=VERTEX_POINT('',#224914);
#42377=VERTEX_POINT('',#224918);
#42378=VERTEX_POINT('',#224919);
#42379=VERTEX_POINT('',#224921);
#42380=VERTEX_POINT('',#224923);
#42381=VERTEX_POINT('',#224925);
#42382=VERTEX_POINT('',#224927);
#42383=VERTEX_POINT('',#224929);
#42384=VERTEX_POINT('',#224931);
#42385=VERTEX_POINT('',#224933);
#42386=VERTEX_POINT('',#224935);
#42387=VERTEX_POINT('',#224937);
#42388=VERTEX_POINT('',#224939);
#42389=VERTEX_POINT('',#224943);
#42390=VERTEX_POINT('',#224944);
#42391=VERTEX_POINT('',#224946);
#42392=VERTEX_POINT('',#224948);
#42393=VERTEX_POINT('',#224950);
#42394=VERTEX_POINT('',#224952);
#42395=VERTEX_POINT('',#224954);
#42396=VERTEX_POINT('',#224956);
#42397=VERTEX_POINT('',#224958);
#42398=VERTEX_POINT('',#224960);
#42399=VERTEX_POINT('',#224962);
#42400=VERTEX_POINT('',#224964);
#42401=VERTEX_POINT('',#225384);
#42402=VERTEX_POINT('',#225385);
#42403=VERTEX_POINT('',#225387);
#42404=VERTEX_POINT('',#225389);
#42405=VERTEX_POINT('',#225393);
#42406=VERTEX_POINT('',#225394);
#42407=VERTEX_POINT('',#225396);
#42408=VERTEX_POINT('',#225398);
#42409=VERTEX_POINT('',#225400);
#42410=VERTEX_POINT('',#225402);
#42411=VERTEX_POINT('',#225404);
#42412=VERTEX_POINT('',#225406);
#42413=VERTEX_POINT('',#225408);
#42414=VERTEX_POINT('',#225410);
#42415=VERTEX_POINT('',#225412);
#42416=VERTEX_POINT('',#225414);
#42417=VERTEX_POINT('',#225418);
#42418=VERTEX_POINT('',#225419);
#42419=VERTEX_POINT('',#225421);
#42420=VERTEX_POINT('',#225423);
#42421=VERTEX_POINT('',#225425);
#42422=VERTEX_POINT('',#225427);
#42423=VERTEX_POINT('',#225429);
#42424=VERTEX_POINT('',#225431);
#42425=VERTEX_POINT('',#225433);
#42426=VERTEX_POINT('',#225435);
#42427=VERTEX_POINT('',#225437);
#42428=VERTEX_POINT('',#225439);
#42429=VERTEX_POINT('',#225443);
#42430=VERTEX_POINT('',#225444);
#42431=VERTEX_POINT('',#225446);
#42432=VERTEX_POINT('',#225448);
#42433=VERTEX_POINT('',#225452);
#42434=VERTEX_POINT('',#225453);
#42435=VERTEX_POINT('',#225455);
#42436=VERTEX_POINT('',#225457);
#42437=VERTEX_POINT('',#225459);
#42438=VERTEX_POINT('',#225461);
#42439=VERTEX_POINT('',#225463);
#42440=VERTEX_POINT('',#225465);
#42441=VERTEX_POINT('',#225467);
#42442=VERTEX_POINT('',#225469);
#42443=VERTEX_POINT('',#225471);
#42444=VERTEX_POINT('',#225473);
#42445=VERTEX_POINT('',#225477);
#42446=VERTEX_POINT('',#225478);
#42447=VERTEX_POINT('',#225480);
#42448=VERTEX_POINT('',#225482);
#42449=VERTEX_POINT('',#225484);
#42450=VERTEX_POINT('',#225486);
#42451=VERTEX_POINT('',#225488);
#42452=VERTEX_POINT('',#225490);
#42453=VERTEX_POINT('',#225492);
#42454=VERTEX_POINT('',#225494);
#42455=VERTEX_POINT('',#225496);
#42456=VERTEX_POINT('',#225498);
#42457=VERTEX_POINT('',#225502);
#42458=VERTEX_POINT('',#225503);
#42459=VERTEX_POINT('',#225505);
#42460=VERTEX_POINT('',#225507);
#42461=VERTEX_POINT('',#225511);
#42462=VERTEX_POINT('',#225512);
#42463=VERTEX_POINT('',#225514);
#42464=VERTEX_POINT('',#225516);
#42465=VERTEX_POINT('',#225518);
#42466=VERTEX_POINT('',#225520);
#42467=VERTEX_POINT('',#225522);
#42468=VERTEX_POINT('',#225524);
#42469=VERTEX_POINT('',#225526);
#42470=VERTEX_POINT('',#225528);
#42471=VERTEX_POINT('',#225530);
#42472=VERTEX_POINT('',#225532);
#42473=VERTEX_POINT('',#225536);
#42474=VERTEX_POINT('',#225537);
#42475=VERTEX_POINT('',#225539);
#42476=VERTEX_POINT('',#225541);
#42477=VERTEX_POINT('',#225543);
#42478=VERTEX_POINT('',#225545);
#42479=VERTEX_POINT('',#225547);
#42480=VERTEX_POINT('',#225549);
#42481=VERTEX_POINT('',#225551);
#42482=VERTEX_POINT('',#225553);
#42483=VERTEX_POINT('',#225555);
#42484=VERTEX_POINT('',#225557);
#42485=VERTEX_POINT('',#225561);
#42486=VERTEX_POINT('',#225562);
#42487=VERTEX_POINT('',#225564);
#42488=VERTEX_POINT('',#225566);
#42489=VERTEX_POINT('',#225570);
#42490=VERTEX_POINT('',#225571);
#42491=VERTEX_POINT('',#225573);
#42492=VERTEX_POINT('',#225575);
#42493=VERTEX_POINT('',#225577);
#42494=VERTEX_POINT('',#225579);
#42495=VERTEX_POINT('',#225581);
#42496=VERTEX_POINT('',#225583);
#42497=VERTEX_POINT('',#225585);
#42498=VERTEX_POINT('',#225587);
#42499=VERTEX_POINT('',#225589);
#42500=VERTEX_POINT('',#225591);
#42501=VERTEX_POINT('',#225595);
#42502=VERTEX_POINT('',#225596);
#42503=VERTEX_POINT('',#225598);
#42504=VERTEX_POINT('',#225600);
#42505=VERTEX_POINT('',#225602);
#42506=VERTEX_POINT('',#225604);
#42507=VERTEX_POINT('',#225606);
#42508=VERTEX_POINT('',#225608);
#42509=VERTEX_POINT('',#225610);
#42510=VERTEX_POINT('',#225612);
#42511=VERTEX_POINT('',#225614);
#42512=VERTEX_POINT('',#225616);
#42513=VERTEX_POINT('',#225620);
#42514=VERTEX_POINT('',#225621);
#42515=VERTEX_POINT('',#225623);
#42516=VERTEX_POINT('',#225625);
#42517=VERTEX_POINT('',#225629);
#42518=VERTEX_POINT('',#225630);
#42519=VERTEX_POINT('',#225632);
#42520=VERTEX_POINT('',#225634);
#42521=VERTEX_POINT('',#225636);
#42522=VERTEX_POINT('',#225638);
#42523=VERTEX_POINT('',#225640);
#42524=VERTEX_POINT('',#225642);
#42525=VERTEX_POINT('',#225644);
#42526=VERTEX_POINT('',#225646);
#42527=VERTEX_POINT('',#225648);
#42528=VERTEX_POINT('',#225650);
#42529=VERTEX_POINT('',#225654);
#42530=VERTEX_POINT('',#225655);
#42531=VERTEX_POINT('',#225657);
#42532=VERTEX_POINT('',#225659);
#42533=VERTEX_POINT('',#225661);
#42534=VERTEX_POINT('',#225663);
#42535=VERTEX_POINT('',#225665);
#42536=VERTEX_POINT('',#225667);
#42537=VERTEX_POINT('',#225669);
#42538=VERTEX_POINT('',#225671);
#42539=VERTEX_POINT('',#225673);
#42540=VERTEX_POINT('',#225675);
#42541=VERTEX_POINT('',#225679);
#42542=VERTEX_POINT('',#225680);
#42543=VERTEX_POINT('',#225682);
#42544=VERTEX_POINT('',#225684);
#42545=VERTEX_POINT('',#225688);
#42546=VERTEX_POINT('',#225689);
#42547=VERTEX_POINT('',#225691);
#42548=VERTEX_POINT('',#225693);
#42549=VERTEX_POINT('',#225695);
#42550=VERTEX_POINT('',#225697);
#42551=VERTEX_POINT('',#225699);
#42552=VERTEX_POINT('',#225701);
#42553=VERTEX_POINT('',#225703);
#42554=VERTEX_POINT('',#225705);
#42555=VERTEX_POINT('',#225707);
#42556=VERTEX_POINT('',#225709);
#42557=VERTEX_POINT('',#225713);
#42558=VERTEX_POINT('',#225714);
#42559=VERTEX_POINT('',#225716);
#42560=VERTEX_POINT('',#225718);
#42561=VERTEX_POINT('',#225720);
#42562=VERTEX_POINT('',#225722);
#42563=VERTEX_POINT('',#225724);
#42564=VERTEX_POINT('',#225726);
#42565=VERTEX_POINT('',#225728);
#42566=VERTEX_POINT('',#225730);
#42567=VERTEX_POINT('',#225732);
#42568=VERTEX_POINT('',#225734);
#42569=VERTEX_POINT('',#225738);
#42570=VERTEX_POINT('',#225739);
#42571=VERTEX_POINT('',#225741);
#42572=VERTEX_POINT('',#225743);
#42573=VERTEX_POINT('',#225747);
#42574=VERTEX_POINT('',#225748);
#42575=VERTEX_POINT('',#225750);
#42576=VERTEX_POINT('',#225752);
#42577=VERTEX_POINT('',#225754);
#42578=VERTEX_POINT('',#225756);
#42579=VERTEX_POINT('',#225758);
#42580=VERTEX_POINT('',#225760);
#42581=VERTEX_POINT('',#225762);
#42582=VERTEX_POINT('',#225764);
#42583=VERTEX_POINT('',#225766);
#42584=VERTEX_POINT('',#225768);
#42585=VERTEX_POINT('',#225772);
#42586=VERTEX_POINT('',#225773);
#42587=VERTEX_POINT('',#225775);
#42588=VERTEX_POINT('',#225777);
#42589=VERTEX_POINT('',#225779);
#42590=VERTEX_POINT('',#225781);
#42591=VERTEX_POINT('',#225783);
#42592=VERTEX_POINT('',#225785);
#42593=VERTEX_POINT('',#225787);
#42594=VERTEX_POINT('',#225789);
#42595=VERTEX_POINT('',#225791);
#42596=VERTEX_POINT('',#225793);
#42597=VERTEX_POINT('',#225797);
#42598=VERTEX_POINT('',#225798);
#42599=VERTEX_POINT('',#225800);
#42600=VERTEX_POINT('',#225802);
#42601=VERTEX_POINT('',#225806);
#42602=VERTEX_POINT('',#225807);
#42603=VERTEX_POINT('',#225809);
#42604=VERTEX_POINT('',#225811);
#42605=VERTEX_POINT('',#225813);
#42606=VERTEX_POINT('',#225815);
#42607=VERTEX_POINT('',#225817);
#42608=VERTEX_POINT('',#225819);
#42609=VERTEX_POINT('',#225821);
#42610=VERTEX_POINT('',#225823);
#42611=VERTEX_POINT('',#225825);
#42612=VERTEX_POINT('',#225827);
#42613=VERTEX_POINT('',#225831);
#42614=VERTEX_POINT('',#225832);
#42615=VERTEX_POINT('',#225834);
#42616=VERTEX_POINT('',#225836);
#42617=VERTEX_POINT('',#225838);
#42618=VERTEX_POINT('',#225840);
#42619=VERTEX_POINT('',#225842);
#42620=VERTEX_POINT('',#225844);
#42621=VERTEX_POINT('',#225846);
#42622=VERTEX_POINT('',#225848);
#42623=VERTEX_POINT('',#225850);
#42624=VERTEX_POINT('',#225852);
#42625=VERTEX_POINT('',#225856);
#42626=VERTEX_POINT('',#225857);
#42627=VERTEX_POINT('',#225859);
#42628=VERTEX_POINT('',#225861);
#42629=VERTEX_POINT('',#225865);
#42630=VERTEX_POINT('',#225866);
#42631=VERTEX_POINT('',#225868);
#42632=VERTEX_POINT('',#225870);
#42633=VERTEX_POINT('',#225872);
#42634=VERTEX_POINT('',#225874);
#42635=VERTEX_POINT('',#225876);
#42636=VERTEX_POINT('',#225878);
#42637=VERTEX_POINT('',#225880);
#42638=VERTEX_POINT('',#225882);
#42639=VERTEX_POINT('',#225884);
#42640=VERTEX_POINT('',#225886);
#42641=VERTEX_POINT('',#225890);
#42642=VERTEX_POINT('',#225891);
#42643=VERTEX_POINT('',#225893);
#42644=VERTEX_POINT('',#225895);
#42645=VERTEX_POINT('',#225897);
#42646=VERTEX_POINT('',#225899);
#42647=VERTEX_POINT('',#225901);
#42648=VERTEX_POINT('',#225903);
#42649=VERTEX_POINT('',#225905);
#42650=VERTEX_POINT('',#225907);
#42651=VERTEX_POINT('',#225909);
#42652=VERTEX_POINT('',#225911);
#42653=VERTEX_POINT('',#225915);
#42654=VERTEX_POINT('',#225916);
#42655=VERTEX_POINT('',#225918);
#42656=VERTEX_POINT('',#225920);
#42657=VERTEX_POINT('',#225924);
#42658=VERTEX_POINT('',#225925);
#42659=VERTEX_POINT('',#225927);
#42660=VERTEX_POINT('',#225929);
#42661=VERTEX_POINT('',#225931);
#42662=VERTEX_POINT('',#225933);
#42663=VERTEX_POINT('',#225935);
#42664=VERTEX_POINT('',#225937);
#42665=VERTEX_POINT('',#225939);
#42666=VERTEX_POINT('',#225941);
#42667=VERTEX_POINT('',#225943);
#42668=VERTEX_POINT('',#225945);
#42669=VERTEX_POINT('',#225949);
#42670=VERTEX_POINT('',#225950);
#42671=VERTEX_POINT('',#225952);
#42672=VERTEX_POINT('',#225954);
#42673=VERTEX_POINT('',#225956);
#42674=VERTEX_POINT('',#225958);
#42675=VERTEX_POINT('',#225960);
#42676=VERTEX_POINT('',#225962);
#42677=VERTEX_POINT('',#225964);
#42678=VERTEX_POINT('',#225966);
#42679=VERTEX_POINT('',#225968);
#42680=VERTEX_POINT('',#225970);
#42681=VERTEX_POINT('',#225974);
#42682=VERTEX_POINT('',#225975);
#42683=VERTEX_POINT('',#225977);
#42684=VERTEX_POINT('',#225979);
#42685=VERTEX_POINT('',#225983);
#42686=VERTEX_POINT('',#225984);
#42687=VERTEX_POINT('',#225986);
#42688=VERTEX_POINT('',#225988);
#42689=VERTEX_POINT('',#225990);
#42690=VERTEX_POINT('',#225992);
#42691=VERTEX_POINT('',#225994);
#42692=VERTEX_POINT('',#225996);
#42693=VERTEX_POINT('',#225998);
#42694=VERTEX_POINT('',#226000);
#42695=VERTEX_POINT('',#226002);
#42696=VERTEX_POINT('',#226004);
#42697=VERTEX_POINT('',#226008);
#42698=VERTEX_POINT('',#226009);
#42699=VERTEX_POINT('',#226011);
#42700=VERTEX_POINT('',#226013);
#42701=VERTEX_POINT('',#226015);
#42702=VERTEX_POINT('',#226017);
#42703=VERTEX_POINT('',#226019);
#42704=VERTEX_POINT('',#226021);
#42705=VERTEX_POINT('',#226023);
#42706=VERTEX_POINT('',#226025);
#42707=VERTEX_POINT('',#226027);
#42708=VERTEX_POINT('',#226029);
#42709=VERTEX_POINT('',#226033);
#42710=VERTEX_POINT('',#226034);
#42711=VERTEX_POINT('',#226036);
#42712=VERTEX_POINT('',#226038);
#42713=VERTEX_POINT('',#226042);
#42714=VERTEX_POINT('',#226043);
#42715=VERTEX_POINT('',#226045);
#42716=VERTEX_POINT('',#226047);
#42717=VERTEX_POINT('',#226049);
#42718=VERTEX_POINT('',#226051);
#42719=VERTEX_POINT('',#226053);
#42720=VERTEX_POINT('',#226055);
#42721=VERTEX_POINT('',#226057);
#42722=VERTEX_POINT('',#226059);
#42723=VERTEX_POINT('',#226061);
#42724=VERTEX_POINT('',#226063);
#42725=VERTEX_POINT('',#226067);
#42726=VERTEX_POINT('',#226068);
#42727=VERTEX_POINT('',#226070);
#42728=VERTEX_POINT('',#226072);
#42729=VERTEX_POINT('',#226074);
#42730=VERTEX_POINT('',#226076);
#42731=VERTEX_POINT('',#226078);
#42732=VERTEX_POINT('',#226080);
#42733=VERTEX_POINT('',#226082);
#42734=VERTEX_POINT('',#226084);
#42735=VERTEX_POINT('',#226086);
#42736=VERTEX_POINT('',#226088);
#42737=VERTEX_POINT('',#226092);
#42738=VERTEX_POINT('',#226093);
#42739=VERTEX_POINT('',#226095);
#42740=VERTEX_POINT('',#226097);
#42741=VERTEX_POINT('',#226101);
#42742=VERTEX_POINT('',#226102);
#42743=VERTEX_POINT('',#226104);
#42744=VERTEX_POINT('',#226106);
#42745=VERTEX_POINT('',#226108);
#42746=VERTEX_POINT('',#226110);
#42747=VERTEX_POINT('',#226112);
#42748=VERTEX_POINT('',#226114);
#42749=VERTEX_POINT('',#226116);
#42750=VERTEX_POINT('',#226118);
#42751=VERTEX_POINT('',#226120);
#42752=VERTEX_POINT('',#226122);
#42753=VERTEX_POINT('',#226126);
#42754=VERTEX_POINT('',#226127);
#42755=VERTEX_POINT('',#226129);
#42756=VERTEX_POINT('',#226131);
#42757=VERTEX_POINT('',#226133);
#42758=VERTEX_POINT('',#226135);
#42759=VERTEX_POINT('',#226137);
#42760=VERTEX_POINT('',#226139);
#42761=VERTEX_POINT('',#226141);
#42762=VERTEX_POINT('',#226143);
#42763=VERTEX_POINT('',#226145);
#42764=VERTEX_POINT('',#226147);
#42765=VERTEX_POINT('',#226151);
#42766=VERTEX_POINT('',#226152);
#42767=VERTEX_POINT('',#226154);
#42768=VERTEX_POINT('',#226156);
#42769=VERTEX_POINT('',#226160);
#42770=VERTEX_POINT('',#226161);
#42771=VERTEX_POINT('',#226163);
#42772=VERTEX_POINT('',#226165);
#42773=VERTEX_POINT('',#226167);
#42774=VERTEX_POINT('',#226169);
#42775=VERTEX_POINT('',#226171);
#42776=VERTEX_POINT('',#226173);
#42777=VERTEX_POINT('',#226175);
#42778=VERTEX_POINT('',#226177);
#42779=VERTEX_POINT('',#226179);
#42780=VERTEX_POINT('',#226181);
#42781=VERTEX_POINT('',#226185);
#42782=VERTEX_POINT('',#226186);
#42783=VERTEX_POINT('',#226188);
#42784=VERTEX_POINT('',#226190);
#42785=VERTEX_POINT('',#226192);
#42786=VERTEX_POINT('',#226194);
#42787=VERTEX_POINT('',#226196);
#42788=VERTEX_POINT('',#226198);
#42789=VERTEX_POINT('',#226200);
#42790=VERTEX_POINT('',#226202);
#42791=VERTEX_POINT('',#226204);
#42792=VERTEX_POINT('',#226206);
#42793=VERTEX_POINT('',#226210);
#42794=VERTEX_POINT('',#226211);
#42795=VERTEX_POINT('',#226213);
#42796=VERTEX_POINT('',#226215);
#42797=VERTEX_POINT('',#226219);
#42798=VERTEX_POINT('',#226220);
#42799=VERTEX_POINT('',#226222);
#42800=VERTEX_POINT('',#226224);
#42801=VERTEX_POINT('',#226226);
#42802=VERTEX_POINT('',#226228);
#42803=VERTEX_POINT('',#226230);
#42804=VERTEX_POINT('',#226232);
#42805=VERTEX_POINT('',#226234);
#42806=VERTEX_POINT('',#226236);
#42807=VERTEX_POINT('',#226238);
#42808=VERTEX_POINT('',#226240);
#42809=VERTEX_POINT('',#226244);
#42810=VERTEX_POINT('',#226245);
#42811=VERTEX_POINT('',#226247);
#42812=VERTEX_POINT('',#226249);
#42813=VERTEX_POINT('',#226251);
#42814=VERTEX_POINT('',#226253);
#42815=VERTEX_POINT('',#226255);
#42816=VERTEX_POINT('',#226257);
#42817=VERTEX_POINT('',#226259);
#42818=VERTEX_POINT('',#226261);
#42819=VERTEX_POINT('',#226263);
#42820=VERTEX_POINT('',#226265);
#42821=VERTEX_POINT('',#226269);
#42822=VERTEX_POINT('',#226270);
#42823=VERTEX_POINT('',#226272);
#42824=VERTEX_POINT('',#226274);
#42825=VERTEX_POINT('',#226278);
#42826=VERTEX_POINT('',#226279);
#42827=VERTEX_POINT('',#226281);
#42828=VERTEX_POINT('',#226283);
#42829=VERTEX_POINT('',#226285);
#42830=VERTEX_POINT('',#226287);
#42831=VERTEX_POINT('',#226289);
#42832=VERTEX_POINT('',#226291);
#42833=VERTEX_POINT('',#226293);
#42834=VERTEX_POINT('',#226295);
#42835=VERTEX_POINT('',#226297);
#42836=VERTEX_POINT('',#226299);
#42837=VERTEX_POINT('',#226303);
#42838=VERTEX_POINT('',#226304);
#42839=VERTEX_POINT('',#226306);
#42840=VERTEX_POINT('',#226308);
#42841=VERTEX_POINT('',#226310);
#42842=VERTEX_POINT('',#226312);
#42843=VERTEX_POINT('',#226314);
#42844=VERTEX_POINT('',#226316);
#42845=VERTEX_POINT('',#226318);
#42846=VERTEX_POINT('',#226320);
#42847=VERTEX_POINT('',#226322);
#42848=VERTEX_POINT('',#226324);
#42849=VERTEX_POINT('',#226328);
#42850=VERTEX_POINT('',#226329);
#42851=VERTEX_POINT('',#226331);
#42852=VERTEX_POINT('',#226333);
#42853=VERTEX_POINT('',#226337);
#42854=VERTEX_POINT('',#226338);
#42855=VERTEX_POINT('',#226340);
#42856=VERTEX_POINT('',#226342);
#42857=VERTEX_POINT('',#226344);
#42858=VERTEX_POINT('',#226346);
#42859=VERTEX_POINT('',#226348);
#42860=VERTEX_POINT('',#226350);
#42861=VERTEX_POINT('',#226352);
#42862=VERTEX_POINT('',#226354);
#42863=VERTEX_POINT('',#226356);
#42864=VERTEX_POINT('',#226358);
#42865=VERTEX_POINT('',#226362);
#42866=VERTEX_POINT('',#226363);
#42867=VERTEX_POINT('',#226365);
#42868=VERTEX_POINT('',#226367);
#42869=VERTEX_POINT('',#226369);
#42870=VERTEX_POINT('',#226371);
#42871=VERTEX_POINT('',#226373);
#42872=VERTEX_POINT('',#226375);
#42873=VERTEX_POINT('',#226377);
#42874=VERTEX_POINT('',#226379);
#42875=VERTEX_POINT('',#226381);
#42876=VERTEX_POINT('',#226383);
#42877=VERTEX_POINT('',#226387);
#42878=VERTEX_POINT('',#226388);
#42879=VERTEX_POINT('',#226390);
#42880=VERTEX_POINT('',#226392);
#42881=VERTEX_POINT('',#226396);
#42882=VERTEX_POINT('',#226397);
#42883=VERTEX_POINT('',#226399);
#42884=VERTEX_POINT('',#226401);
#42885=VERTEX_POINT('',#226403);
#42886=VERTEX_POINT('',#226405);
#42887=VERTEX_POINT('',#226407);
#42888=VERTEX_POINT('',#226409);
#42889=VERTEX_POINT('',#226411);
#42890=VERTEX_POINT('',#226413);
#42891=VERTEX_POINT('',#226415);
#42892=VERTEX_POINT('',#226417);
#42893=VERTEX_POINT('',#226421);
#42894=VERTEX_POINT('',#226422);
#42895=VERTEX_POINT('',#226424);
#42896=VERTEX_POINT('',#226426);
#42897=VERTEX_POINT('',#226428);
#42898=VERTEX_POINT('',#226430);
#42899=VERTEX_POINT('',#226432);
#42900=VERTEX_POINT('',#226434);
#42901=VERTEX_POINT('',#226436);
#42902=VERTEX_POINT('',#226438);
#42903=VERTEX_POINT('',#226440);
#42904=VERTEX_POINT('',#226442);
#42905=VERTEX_POINT('',#226446);
#42906=VERTEX_POINT('',#226447);
#42907=VERTEX_POINT('',#226449);
#42908=VERTEX_POINT('',#226451);
#42909=VERTEX_POINT('',#226455);
#42910=VERTEX_POINT('',#226456);
#42911=VERTEX_POINT('',#226458);
#42912=VERTEX_POINT('',#226460);
#42913=VERTEX_POINT('',#226462);
#42914=VERTEX_POINT('',#226464);
#42915=VERTEX_POINT('',#226466);
#42916=VERTEX_POINT('',#226468);
#42917=VERTEX_POINT('',#226470);
#42918=VERTEX_POINT('',#226472);
#42919=VERTEX_POINT('',#226474);
#42920=VERTEX_POINT('',#226476);
#42921=VERTEX_POINT('',#226480);
#42922=VERTEX_POINT('',#226481);
#42923=VERTEX_POINT('',#226483);
#42924=VERTEX_POINT('',#226485);
#42925=VERTEX_POINT('',#226487);
#42926=VERTEX_POINT('',#226489);
#42927=VERTEX_POINT('',#226491);
#42928=VERTEX_POINT('',#226493);
#42929=VERTEX_POINT('',#226495);
#42930=VERTEX_POINT('',#226497);
#42931=VERTEX_POINT('',#226499);
#42932=VERTEX_POINT('',#226501);
#42933=VERTEX_POINT('',#226505);
#42934=VERTEX_POINT('',#226506);
#42935=VERTEX_POINT('',#226508);
#42936=VERTEX_POINT('',#226510);
#42937=VERTEX_POINT('',#226514);
#42938=VERTEX_POINT('',#226515);
#42939=VERTEX_POINT('',#226517);
#42940=VERTEX_POINT('',#226519);
#42941=VERTEX_POINT('',#226521);
#42942=VERTEX_POINT('',#226523);
#42943=VERTEX_POINT('',#226525);
#42944=VERTEX_POINT('',#226527);
#42945=VERTEX_POINT('',#226529);
#42946=VERTEX_POINT('',#226531);
#42947=VERTEX_POINT('',#226533);
#42948=VERTEX_POINT('',#226535);
#42949=VERTEX_POINT('',#226539);
#42950=VERTEX_POINT('',#226540);
#42951=VERTEX_POINT('',#226542);
#42952=VERTEX_POINT('',#226544);
#42953=VERTEX_POINT('',#226546);
#42954=VERTEX_POINT('',#226548);
#42955=VERTEX_POINT('',#226550);
#42956=VERTEX_POINT('',#226552);
#42957=VERTEX_POINT('',#226554);
#42958=VERTEX_POINT('',#226556);
#42959=VERTEX_POINT('',#226558);
#42960=VERTEX_POINT('',#226560);
#42961=VERTEX_POINT('',#226564);
#42962=VERTEX_POINT('',#226565);
#42963=VERTEX_POINT('',#226567);
#42964=VERTEX_POINT('',#226569);
#42965=VERTEX_POINT('',#226573);
#42966=VERTEX_POINT('',#226574);
#42967=VERTEX_POINT('',#226576);
#42968=VERTEX_POINT('',#226578);
#42969=VERTEX_POINT('',#226580);
#42970=VERTEX_POINT('',#226582);
#42971=VERTEX_POINT('',#226584);
#42972=VERTEX_POINT('',#226586);
#42973=VERTEX_POINT('',#226588);
#42974=VERTEX_POINT('',#226590);
#42975=VERTEX_POINT('',#226592);
#42976=VERTEX_POINT('',#226594);
#42977=VERTEX_POINT('',#226598);
#42978=VERTEX_POINT('',#226599);
#42979=VERTEX_POINT('',#226601);
#42980=VERTEX_POINT('',#226603);
#42981=VERTEX_POINT('',#226605);
#42982=VERTEX_POINT('',#226607);
#42983=VERTEX_POINT('',#226609);
#42984=VERTEX_POINT('',#226611);
#42985=VERTEX_POINT('',#226613);
#42986=VERTEX_POINT('',#226615);
#42987=VERTEX_POINT('',#226617);
#42988=VERTEX_POINT('',#226619);
#42989=VERTEX_POINT('',#226623);
#42990=VERTEX_POINT('',#226624);
#42991=VERTEX_POINT('',#226626);
#42992=VERTEX_POINT('',#226628);
#42993=VERTEX_POINT('',#226632);
#42994=VERTEX_POINT('',#226633);
#42995=VERTEX_POINT('',#226635);
#42996=VERTEX_POINT('',#226637);
#42997=VERTEX_POINT('',#226639);
#42998=VERTEX_POINT('',#226641);
#42999=VERTEX_POINT('',#226643);
#43000=VERTEX_POINT('',#226645);
#43001=VERTEX_POINT('',#226647);
#43002=VERTEX_POINT('',#226649);
#43003=VERTEX_POINT('',#226651);
#43004=VERTEX_POINT('',#226653);
#43005=VERTEX_POINT('',#226657);
#43006=VERTEX_POINT('',#226658);
#43007=VERTEX_POINT('',#226660);
#43008=VERTEX_POINT('',#226662);
#43009=VERTEX_POINT('',#226664);
#43010=VERTEX_POINT('',#226666);
#43011=VERTEX_POINT('',#226668);
#43012=VERTEX_POINT('',#226670);
#43013=VERTEX_POINT('',#226672);
#43014=VERTEX_POINT('',#226674);
#43015=VERTEX_POINT('',#226676);
#43016=VERTEX_POINT('',#226678);
#43017=VERTEX_POINT('',#226682);
#43018=VERTEX_POINT('',#226683);
#43019=VERTEX_POINT('',#226685);
#43020=VERTEX_POINT('',#226687);
#43021=VERTEX_POINT('',#226691);
#43022=VERTEX_POINT('',#226692);
#43023=VERTEX_POINT('',#226694);
#43024=VERTEX_POINT('',#226696);
#43025=VERTEX_POINT('',#226698);
#43026=VERTEX_POINT('',#226700);
#43027=VERTEX_POINT('',#226702);
#43028=VERTEX_POINT('',#226704);
#43029=VERTEX_POINT('',#226706);
#43030=VERTEX_POINT('',#226708);
#43031=VERTEX_POINT('',#226710);
#43032=VERTEX_POINT('',#226712);
#43033=VERTEX_POINT('',#226716);
#43034=VERTEX_POINT('',#226717);
#43035=VERTEX_POINT('',#226719);
#43036=VERTEX_POINT('',#226721);
#43037=VERTEX_POINT('',#226723);
#43038=VERTEX_POINT('',#226725);
#43039=VERTEX_POINT('',#226727);
#43040=VERTEX_POINT('',#226729);
#43041=VERTEX_POINT('',#226731);
#43042=VERTEX_POINT('',#226733);
#43043=VERTEX_POINT('',#226735);
#43044=VERTEX_POINT('',#226737);
#43045=VERTEX_POINT('',#226741);
#43046=VERTEX_POINT('',#226742);
#43047=VERTEX_POINT('',#226744);
#43048=VERTEX_POINT('',#226746);
#43049=VERTEX_POINT('',#226750);
#43050=VERTEX_POINT('',#226751);
#43051=VERTEX_POINT('',#226753);
#43052=VERTEX_POINT('',#226755);
#43053=VERTEX_POINT('',#226757);
#43054=VERTEX_POINT('',#226759);
#43055=VERTEX_POINT('',#226761);
#43056=VERTEX_POINT('',#226763);
#43057=VERTEX_POINT('',#226765);
#43058=VERTEX_POINT('',#226767);
#43059=VERTEX_POINT('',#226769);
#43060=VERTEX_POINT('',#226771);
#43061=VERTEX_POINT('',#226775);
#43062=VERTEX_POINT('',#226776);
#43063=VERTEX_POINT('',#226778);
#43064=VERTEX_POINT('',#226780);
#43065=VERTEX_POINT('',#226782);
#43066=VERTEX_POINT('',#226784);
#43067=VERTEX_POINT('',#226786);
#43068=VERTEX_POINT('',#226788);
#43069=VERTEX_POINT('',#226790);
#43070=VERTEX_POINT('',#226792);
#43071=VERTEX_POINT('',#226794);
#43072=VERTEX_POINT('',#226796);
#43073=VERTEX_POINT('',#226800);
#43074=VERTEX_POINT('',#226801);
#43075=VERTEX_POINT('',#226803);
#43076=VERTEX_POINT('',#226805);
#43077=VERTEX_POINT('',#226809);
#43078=VERTEX_POINT('',#226810);
#43079=VERTEX_POINT('',#226812);
#43080=VERTEX_POINT('',#226814);
#43081=VERTEX_POINT('',#226816);
#43082=VERTEX_POINT('',#226818);
#43083=VERTEX_POINT('',#226820);
#43084=VERTEX_POINT('',#226822);
#43085=VERTEX_POINT('',#226824);
#43086=VERTEX_POINT('',#226826);
#43087=VERTEX_POINT('',#226828);
#43088=VERTEX_POINT('',#226830);
#43089=VERTEX_POINT('',#226834);
#43090=VERTEX_POINT('',#226835);
#43091=VERTEX_POINT('',#226837);
#43092=VERTEX_POINT('',#226839);
#43093=VERTEX_POINT('',#226841);
#43094=VERTEX_POINT('',#226843);
#43095=VERTEX_POINT('',#226845);
#43096=VERTEX_POINT('',#226847);
#43097=VERTEX_POINT('',#226849);
#43098=VERTEX_POINT('',#226851);
#43099=VERTEX_POINT('',#226853);
#43100=VERTEX_POINT('',#226855);
#43101=VERTEX_POINT('',#226859);
#43102=VERTEX_POINT('',#226860);
#43103=VERTEX_POINT('',#226862);
#43104=VERTEX_POINT('',#226864);
#43105=VERTEX_POINT('',#226868);
#43106=VERTEX_POINT('',#226869);
#43107=VERTEX_POINT('',#226871);
#43108=VERTEX_POINT('',#226873);
#43109=VERTEX_POINT('',#226875);
#43110=VERTEX_POINT('',#226877);
#43111=VERTEX_POINT('',#226879);
#43112=VERTEX_POINT('',#226881);
#43113=VERTEX_POINT('',#226883);
#43114=VERTEX_POINT('',#226885);
#43115=VERTEX_POINT('',#226887);
#43116=VERTEX_POINT('',#226889);
#43117=VERTEX_POINT('',#226893);
#43118=VERTEX_POINT('',#226894);
#43119=VERTEX_POINT('',#226896);
#43120=VERTEX_POINT('',#226898);
#43121=VERTEX_POINT('',#226900);
#43122=VERTEX_POINT('',#226902);
#43123=VERTEX_POINT('',#226904);
#43124=VERTEX_POINT('',#226906);
#43125=VERTEX_POINT('',#226908);
#43126=VERTEX_POINT('',#226910);
#43127=VERTEX_POINT('',#226912);
#43128=VERTEX_POINT('',#226914);
#43129=VERTEX_POINT('',#226918);
#43130=VERTEX_POINT('',#226919);
#43131=VERTEX_POINT('',#226921);
#43132=VERTEX_POINT('',#226923);
#43133=VERTEX_POINT('',#226927);
#43134=VERTEX_POINT('',#226928);
#43135=VERTEX_POINT('',#226930);
#43136=VERTEX_POINT('',#226932);
#43137=VERTEX_POINT('',#226934);
#43138=VERTEX_POINT('',#226936);
#43139=VERTEX_POINT('',#226938);
#43140=VERTEX_POINT('',#226940);
#43141=VERTEX_POINT('',#226942);
#43142=VERTEX_POINT('',#226944);
#43143=VERTEX_POINT('',#226946);
#43144=VERTEX_POINT('',#226948);
#43145=VERTEX_POINT('',#226952);
#43146=VERTEX_POINT('',#226953);
#43147=VERTEX_POINT('',#226955);
#43148=VERTEX_POINT('',#226957);
#43149=VERTEX_POINT('',#226959);
#43150=VERTEX_POINT('',#226961);
#43151=VERTEX_POINT('',#226963);
#43152=VERTEX_POINT('',#226965);
#43153=VERTEX_POINT('',#226967);
#43154=VERTEX_POINT('',#226969);
#43155=VERTEX_POINT('',#226971);
#43156=VERTEX_POINT('',#226973);
#43157=VERTEX_POINT('',#226977);
#43158=VERTEX_POINT('',#226978);
#43159=VERTEX_POINT('',#226980);
#43160=VERTEX_POINT('',#226982);
#43161=VERTEX_POINT('',#226986);
#43162=VERTEX_POINT('',#226987);
#43163=VERTEX_POINT('',#226989);
#43164=VERTEX_POINT('',#226991);
#43165=VERTEX_POINT('',#226993);
#43166=VERTEX_POINT('',#226995);
#43167=VERTEX_POINT('',#226997);
#43168=VERTEX_POINT('',#226999);
#43169=VERTEX_POINT('',#227001);
#43170=VERTEX_POINT('',#227003);
#43171=VERTEX_POINT('',#227005);
#43172=VERTEX_POINT('',#227007);
#43173=VERTEX_POINT('',#227011);
#43174=VERTEX_POINT('',#227012);
#43175=VERTEX_POINT('',#227014);
#43176=VERTEX_POINT('',#227016);
#43177=VERTEX_POINT('',#227018);
#43178=VERTEX_POINT('',#227020);
#43179=VERTEX_POINT('',#227022);
#43180=VERTEX_POINT('',#227024);
#43181=VERTEX_POINT('',#227026);
#43182=VERTEX_POINT('',#227028);
#43183=VERTEX_POINT('',#227030);
#43184=VERTEX_POINT('',#227032);
#43185=VERTEX_POINT('',#227036);
#43186=VERTEX_POINT('',#227037);
#43187=VERTEX_POINT('',#227039);
#43188=VERTEX_POINT('',#227041);
#43189=VERTEX_POINT('',#227045);
#43190=VERTEX_POINT('',#227046);
#43191=VERTEX_POINT('',#227048);
#43192=VERTEX_POINT('',#227050);
#43193=VERTEX_POINT('',#227052);
#43194=VERTEX_POINT('',#227054);
#43195=VERTEX_POINT('',#227056);
#43196=VERTEX_POINT('',#227058);
#43197=VERTEX_POINT('',#227060);
#43198=VERTEX_POINT('',#227062);
#43199=VERTEX_POINT('',#227064);
#43200=VERTEX_POINT('',#227066);
#43201=VERTEX_POINT('',#227070);
#43202=VERTEX_POINT('',#227071);
#43203=VERTEX_POINT('',#227073);
#43204=VERTEX_POINT('',#227075);
#43205=VERTEX_POINT('',#227077);
#43206=VERTEX_POINT('',#227079);
#43207=VERTEX_POINT('',#227081);
#43208=VERTEX_POINT('',#227083);
#43209=VERTEX_POINT('',#227085);
#43210=VERTEX_POINT('',#227087);
#43211=VERTEX_POINT('',#227089);
#43212=VERTEX_POINT('',#227091);
#43213=VERTEX_POINT('',#227098);
#43214=VERTEX_POINT('',#227099);
#43215=VERTEX_POINT('',#227101);
#43216=VERTEX_POINT('',#227103);
#43217=VERTEX_POINT('',#227105);
#43218=VERTEX_POINT('',#227107);
#43219=VERTEX_POINT('',#227109);
#43220=VERTEX_POINT('',#227111);
#43221=VERTEX_POINT('',#227113);
#43222=VERTEX_POINT('',#227115);
#43223=VERTEX_POINT('',#227117);
#43224=VERTEX_POINT('',#227119);
#43225=VERTEX_POINT('',#227123);
#43226=VERTEX_POINT('',#227124);
#43227=VERTEX_POINT('',#227126);
#43228=VERTEX_POINT('',#227128);
#43229=VERTEX_POINT('',#227130);
#43230=VERTEX_POINT('',#227132);
#43231=VERTEX_POINT('',#227134);
#43232=VERTEX_POINT('',#227136);
#43233=VERTEX_POINT('',#227138);
#43234=VERTEX_POINT('',#227140);
#43235=VERTEX_POINT('',#227142);
#43236=VERTEX_POINT('',#227144);
#43237=VERTEX_POINT('',#227148);
#43238=VERTEX_POINT('',#227149);
#43239=VERTEX_POINT('',#227151);
#43240=VERTEX_POINT('',#227153);
#43241=VERTEX_POINT('',#227157);
#43242=VERTEX_POINT('',#227158);
#43243=VERTEX_POINT('',#227160);
#43244=VERTEX_POINT('',#227162);
#43245=VERTEX_POINT('',#227164);
#43246=VERTEX_POINT('',#227166);
#43247=VERTEX_POINT('',#227168);
#43248=VERTEX_POINT('',#227170);
#43249=VERTEX_POINT('',#227172);
#43250=VERTEX_POINT('',#227174);
#43251=VERTEX_POINT('',#227176);
#43252=VERTEX_POINT('',#227178);
#43253=VERTEX_POINT('',#227182);
#43254=VERTEX_POINT('',#227183);
#43255=VERTEX_POINT('',#227185);
#43256=VERTEX_POINT('',#227187);
#43257=VERTEX_POINT('',#227189);
#43258=VERTEX_POINT('',#227191);
#43259=VERTEX_POINT('',#227193);
#43260=VERTEX_POINT('',#227195);
#43261=VERTEX_POINT('',#227197);
#43262=VERTEX_POINT('',#227199);
#43263=VERTEX_POINT('',#227201);
#43264=VERTEX_POINT('',#227203);
#43265=VERTEX_POINT('',#227207);
#43266=VERTEX_POINT('',#227208);
#43267=VERTEX_POINT('',#227210);
#43268=VERTEX_POINT('',#227212);
#43269=VERTEX_POINT('',#227216);
#43270=VERTEX_POINT('',#227217);
#43271=VERTEX_POINT('',#227219);
#43272=VERTEX_POINT('',#227221);
#43273=VERTEX_POINT('',#227223);
#43274=VERTEX_POINT('',#227225);
#43275=VERTEX_POINT('',#227227);
#43276=VERTEX_POINT('',#227229);
#43277=VERTEX_POINT('',#227231);
#43278=VERTEX_POINT('',#227233);
#43279=VERTEX_POINT('',#227235);
#43280=VERTEX_POINT('',#227237);
#43281=VERTEX_POINT('',#227241);
#43282=VERTEX_POINT('',#227242);
#43283=VERTEX_POINT('',#227244);
#43284=VERTEX_POINT('',#227246);
#43285=VERTEX_POINT('',#227248);
#43286=VERTEX_POINT('',#227250);
#43287=VERTEX_POINT('',#227252);
#43288=VERTEX_POINT('',#227254);
#43289=VERTEX_POINT('',#227256);
#43290=VERTEX_POINT('',#227258);
#43291=VERTEX_POINT('',#227260);
#43292=VERTEX_POINT('',#227262);
#43293=VERTEX_POINT('',#227266);
#43294=VERTEX_POINT('',#227267);
#43295=VERTEX_POINT('',#227269);
#43296=VERTEX_POINT('',#227271);
#43297=VERTEX_POINT('',#227275);
#43298=VERTEX_POINT('',#227276);
#43299=VERTEX_POINT('',#227278);
#43300=VERTEX_POINT('',#227280);
#43301=VERTEX_POINT('',#227282);
#43302=VERTEX_POINT('',#227284);
#43303=VERTEX_POINT('',#227286);
#43304=VERTEX_POINT('',#227288);
#43305=VERTEX_POINT('',#227290);
#43306=VERTEX_POINT('',#227292);
#43307=VERTEX_POINT('',#227294);
#43308=VERTEX_POINT('',#227296);
#43309=VERTEX_POINT('',#227300);
#43310=VERTEX_POINT('',#227301);
#43311=VERTEX_POINT('',#227303);
#43312=VERTEX_POINT('',#227305);
#43313=VERTEX_POINT('',#227307);
#43314=VERTEX_POINT('',#227309);
#43315=VERTEX_POINT('',#227311);
#43316=VERTEX_POINT('',#227313);
#43317=VERTEX_POINT('',#227315);
#43318=VERTEX_POINT('',#227317);
#43319=VERTEX_POINT('',#227319);
#43320=VERTEX_POINT('',#227321);
#43321=VERTEX_POINT('',#227325);
#43322=VERTEX_POINT('',#227326);
#43323=VERTEX_POINT('',#227328);
#43324=VERTEX_POINT('',#227330);
#43325=VERTEX_POINT('',#227334);
#43326=VERTEX_POINT('',#227335);
#43327=VERTEX_POINT('',#227337);
#43328=VERTEX_POINT('',#227339);
#43329=VERTEX_POINT('',#227341);
#43330=VERTEX_POINT('',#227343);
#43331=VERTEX_POINT('',#227345);
#43332=VERTEX_POINT('',#227347);
#43333=VERTEX_POINT('',#227349);
#43334=VERTEX_POINT('',#227351);
#43335=VERTEX_POINT('',#227353);
#43336=VERTEX_POINT('',#227355);
#43337=VERTEX_POINT('',#227359);
#43338=VERTEX_POINT('',#227360);
#43339=VERTEX_POINT('',#227362);
#43340=VERTEX_POINT('',#227364);
#43341=VERTEX_POINT('',#227366);
#43342=VERTEX_POINT('',#227368);
#43343=VERTEX_POINT('',#227370);
#43344=VERTEX_POINT('',#227372);
#43345=VERTEX_POINT('',#227374);
#43346=VERTEX_POINT('',#227376);
#43347=VERTEX_POINT('',#227378);
#43348=VERTEX_POINT('',#227380);
#43349=VERTEX_POINT('',#227384);
#43350=VERTEX_POINT('',#227385);
#43351=VERTEX_POINT('',#227387);
#43352=VERTEX_POINT('',#227389);
#43353=VERTEX_POINT('',#227393);
#43354=VERTEX_POINT('',#227394);
#43355=VERTEX_POINT('',#227396);
#43356=VERTEX_POINT('',#227398);
#43357=VERTEX_POINT('',#227400);
#43358=VERTEX_POINT('',#227402);
#43359=VERTEX_POINT('',#227404);
#43360=VERTEX_POINT('',#227406);
#43361=VERTEX_POINT('',#227408);
#43362=VERTEX_POINT('',#227410);
#43363=VERTEX_POINT('',#227412);
#43364=VERTEX_POINT('',#227414);
#43365=VERTEX_POINT('',#227418);
#43366=VERTEX_POINT('',#227419);
#43367=VERTEX_POINT('',#227421);
#43368=VERTEX_POINT('',#227423);
#43369=VERTEX_POINT('',#227425);
#43370=VERTEX_POINT('',#227427);
#43371=VERTEX_POINT('',#227429);
#43372=VERTEX_POINT('',#227431);
#43373=VERTEX_POINT('',#227433);
#43374=VERTEX_POINT('',#227435);
#43375=VERTEX_POINT('',#227437);
#43376=VERTEX_POINT('',#227439);
#43377=VERTEX_POINT('',#227443);
#43378=VERTEX_POINT('',#227444);
#43379=VERTEX_POINT('',#227446);
#43380=VERTEX_POINT('',#227448);
#43381=VERTEX_POINT('',#227452);
#43382=VERTEX_POINT('',#227453);
#43383=VERTEX_POINT('',#227455);
#43384=VERTEX_POINT('',#227457);
#43385=VERTEX_POINT('',#227459);
#43386=VERTEX_POINT('',#227461);
#43387=VERTEX_POINT('',#227463);
#43388=VERTEX_POINT('',#227465);
#43389=VERTEX_POINT('',#227467);
#43390=VERTEX_POINT('',#227469);
#43391=VERTEX_POINT('',#227471);
#43392=VERTEX_POINT('',#227473);
#43393=VERTEX_POINT('',#227477);
#43394=VERTEX_POINT('',#227478);
#43395=VERTEX_POINT('',#227480);
#43396=VERTEX_POINT('',#227482);
#43397=VERTEX_POINT('',#227484);
#43398=VERTEX_POINT('',#227486);
#43399=VERTEX_POINT('',#227488);
#43400=VERTEX_POINT('',#227490);
#43401=VERTEX_POINT('',#227492);
#43402=VERTEX_POINT('',#227494);
#43403=VERTEX_POINT('',#227496);
#43404=VERTEX_POINT('',#227498);
#43405=VERTEX_POINT('',#227502);
#43406=VERTEX_POINT('',#227503);
#43407=VERTEX_POINT('',#227505);
#43408=VERTEX_POINT('',#227507);
#43409=VERTEX_POINT('',#227511);
#43410=VERTEX_POINT('',#227512);
#43411=VERTEX_POINT('',#227514);
#43412=VERTEX_POINT('',#227516);
#43413=VERTEX_POINT('',#227518);
#43414=VERTEX_POINT('',#227520);
#43415=VERTEX_POINT('',#227522);
#43416=VERTEX_POINT('',#227524);
#43417=VERTEX_POINT('',#227526);
#43418=VERTEX_POINT('',#227528);
#43419=VERTEX_POINT('',#227530);
#43420=VERTEX_POINT('',#227532);
#43421=VERTEX_POINT('',#227536);
#43422=VERTEX_POINT('',#227537);
#43423=VERTEX_POINT('',#227539);
#43424=VERTEX_POINT('',#227541);
#43425=VERTEX_POINT('',#227543);
#43426=VERTEX_POINT('',#227545);
#43427=VERTEX_POINT('',#227547);
#43428=VERTEX_POINT('',#227549);
#43429=VERTEX_POINT('',#227551);
#43430=VERTEX_POINT('',#227553);
#43431=VERTEX_POINT('',#227555);
#43432=VERTEX_POINT('',#227557);
#43433=VERTEX_POINT('',#227561);
#43434=VERTEX_POINT('',#227562);
#43435=VERTEX_POINT('',#227564);
#43436=VERTEX_POINT('',#227566);
#43437=VERTEX_POINT('',#227570);
#43438=VERTEX_POINT('',#227571);
#43439=VERTEX_POINT('',#227573);
#43440=VERTEX_POINT('',#227575);
#43441=VERTEX_POINT('',#227577);
#43442=VERTEX_POINT('',#227579);
#43443=VERTEX_POINT('',#227581);
#43444=VERTEX_POINT('',#227583);
#43445=VERTEX_POINT('',#227585);
#43446=VERTEX_POINT('',#227587);
#43447=VERTEX_POINT('',#227589);
#43448=VERTEX_POINT('',#227591);
#43449=VERTEX_POINT('',#227595);
#43450=VERTEX_POINT('',#227596);
#43451=VERTEX_POINT('',#227598);
#43452=VERTEX_POINT('',#227600);
#43453=VERTEX_POINT('',#227602);
#43454=VERTEX_POINT('',#227604);
#43455=VERTEX_POINT('',#227606);
#43456=VERTEX_POINT('',#227608);
#43457=VERTEX_POINT('',#227610);
#43458=VERTEX_POINT('',#227612);
#43459=VERTEX_POINT('',#227614);
#43460=VERTEX_POINT('',#227616);
#43461=VERTEX_POINT('',#227620);
#43462=VERTEX_POINT('',#227621);
#43463=VERTEX_POINT('',#227623);
#43464=VERTEX_POINT('',#227625);
#43465=VERTEX_POINT('',#227629);
#43466=VERTEX_POINT('',#227630);
#43467=VERTEX_POINT('',#227632);
#43468=VERTEX_POINT('',#227634);
#43469=VERTEX_POINT('',#227636);
#43470=VERTEX_POINT('',#227638);
#43471=VERTEX_POINT('',#227640);
#43472=VERTEX_POINT('',#227642);
#43473=VERTEX_POINT('',#227644);
#43474=VERTEX_POINT('',#227646);
#43475=VERTEX_POINT('',#227648);
#43476=VERTEX_POINT('',#227650);
#43477=VERTEX_POINT('',#227654);
#43478=VERTEX_POINT('',#227655);
#43479=VERTEX_POINT('',#227657);
#43480=VERTEX_POINT('',#227659);
#43481=VERTEX_POINT('',#227661);
#43482=VERTEX_POINT('',#227663);
#43483=VERTEX_POINT('',#227665);
#43484=VERTEX_POINT('',#227667);
#43485=VERTEX_POINT('',#227669);
#43486=VERTEX_POINT('',#227671);
#43487=VERTEX_POINT('',#227673);
#43488=VERTEX_POINT('',#227675);
#43489=VERTEX_POINT('',#227679);
#43490=VERTEX_POINT('',#227680);
#43491=VERTEX_POINT('',#227682);
#43492=VERTEX_POINT('',#227684);
#43493=VERTEX_POINT('',#227688);
#43494=VERTEX_POINT('',#227689);
#43495=VERTEX_POINT('',#227691);
#43496=VERTEX_POINT('',#227693);
#43497=VERTEX_POINT('',#227695);
#43498=VERTEX_POINT('',#227697);
#43499=VERTEX_POINT('',#227699);
#43500=VERTEX_POINT('',#227701);
#43501=VERTEX_POINT('',#227703);
#43502=VERTEX_POINT('',#227705);
#43503=VERTEX_POINT('',#227707);
#43504=VERTEX_POINT('',#227709);
#43505=VERTEX_POINT('',#227713);
#43506=VERTEX_POINT('',#227714);
#43507=VERTEX_POINT('',#227716);
#43508=VERTEX_POINT('',#227718);
#43509=VERTEX_POINT('',#227720);
#43510=VERTEX_POINT('',#227722);
#43511=VERTEX_POINT('',#227724);
#43512=VERTEX_POINT('',#227726);
#43513=VERTEX_POINT('',#227728);
#43514=VERTEX_POINT('',#227730);
#43515=VERTEX_POINT('',#227732);
#43516=VERTEX_POINT('',#227734);
#43517=VERTEX_POINT('',#227738);
#43518=VERTEX_POINT('',#227739);
#43519=VERTEX_POINT('',#227741);
#43520=VERTEX_POINT('',#227743);
#43521=VERTEX_POINT('',#227747);
#43522=VERTEX_POINT('',#227748);
#43523=VERTEX_POINT('',#227750);
#43524=VERTEX_POINT('',#227752);
#43525=VERTEX_POINT('',#227754);
#43526=VERTEX_POINT('',#227756);
#43527=VERTEX_POINT('',#227758);
#43528=VERTEX_POINT('',#227760);
#43529=VERTEX_POINT('',#227762);
#43530=VERTEX_POINT('',#227764);
#43531=VERTEX_POINT('',#227766);
#43532=VERTEX_POINT('',#227768);
#43533=VERTEX_POINT('',#227772);
#43534=VERTEX_POINT('',#227773);
#43535=VERTEX_POINT('',#227775);
#43536=VERTEX_POINT('',#227777);
#43537=VERTEX_POINT('',#227779);
#43538=VERTEX_POINT('',#227781);
#43539=VERTEX_POINT('',#227783);
#43540=VERTEX_POINT('',#227785);
#43541=VERTEX_POINT('',#227787);
#43542=VERTEX_POINT('',#227789);
#43543=VERTEX_POINT('',#227791);
#43544=VERTEX_POINT('',#227793);
#43545=VERTEX_POINT('',#227797);
#43546=VERTEX_POINT('',#227798);
#43547=VERTEX_POINT('',#227800);
#43548=VERTEX_POINT('',#227802);
#43549=VERTEX_POINT('',#227806);
#43550=VERTEX_POINT('',#227807);
#43551=VERTEX_POINT('',#227809);
#43552=VERTEX_POINT('',#227811);
#43553=VERTEX_POINT('',#227813);
#43554=VERTEX_POINT('',#227815);
#43555=VERTEX_POINT('',#227817);
#43556=VERTEX_POINT('',#227819);
#43557=VERTEX_POINT('',#227821);
#43558=VERTEX_POINT('',#227823);
#43559=VERTEX_POINT('',#227825);
#43560=VERTEX_POINT('',#227827);
#43561=VERTEX_POINT('',#227831);
#43562=VERTEX_POINT('',#227832);
#43563=VERTEX_POINT('',#227834);
#43564=VERTEX_POINT('',#227836);
#43565=VERTEX_POINT('',#227838);
#43566=VERTEX_POINT('',#227840);
#43567=VERTEX_POINT('',#227842);
#43568=VERTEX_POINT('',#227844);
#43569=VERTEX_POINT('',#227846);
#43570=VERTEX_POINT('',#227848);
#43571=VERTEX_POINT('',#227850);
#43572=VERTEX_POINT('',#227852);
#43573=VERTEX_POINT('',#227856);
#43574=VERTEX_POINT('',#227857);
#43575=VERTEX_POINT('',#227859);
#43576=VERTEX_POINT('',#227861);
#43577=VERTEX_POINT('',#227865);
#43578=VERTEX_POINT('',#227866);
#43579=VERTEX_POINT('',#227868);
#43580=VERTEX_POINT('',#227870);
#43581=VERTEX_POINT('',#227872);
#43582=VERTEX_POINT('',#227874);
#43583=VERTEX_POINT('',#227876);
#43584=VERTEX_POINT('',#227878);
#43585=VERTEX_POINT('',#227880);
#43586=VERTEX_POINT('',#227882);
#43587=VERTEX_POINT('',#227884);
#43588=VERTEX_POINT('',#227886);
#43589=VERTEX_POINT('',#227890);
#43590=VERTEX_POINT('',#227891);
#43591=VERTEX_POINT('',#227893);
#43592=VERTEX_POINT('',#227895);
#43593=VERTEX_POINT('',#227897);
#43594=VERTEX_POINT('',#227899);
#43595=VERTEX_POINT('',#227901);
#43596=VERTEX_POINT('',#227903);
#43597=VERTEX_POINT('',#227905);
#43598=VERTEX_POINT('',#227907);
#43599=VERTEX_POINT('',#227909);
#43600=VERTEX_POINT('',#227911);
#43601=VERTEX_POINT('',#227915);
#43602=VERTEX_POINT('',#227916);
#43603=VERTEX_POINT('',#227918);
#43604=VERTEX_POINT('',#227920);
#43605=VERTEX_POINT('',#227924);
#43606=VERTEX_POINT('',#227925);
#43607=VERTEX_POINT('',#227927);
#43608=VERTEX_POINT('',#227929);
#43609=VERTEX_POINT('',#227931);
#43610=VERTEX_POINT('',#227933);
#43611=VERTEX_POINT('',#227935);
#43612=VERTEX_POINT('',#227937);
#43613=VERTEX_POINT('',#227939);
#43614=VERTEX_POINT('',#227941);
#43615=VERTEX_POINT('',#227943);
#43616=VERTEX_POINT('',#227945);
#43617=VERTEX_POINT('',#227949);
#43618=VERTEX_POINT('',#227950);
#43619=VERTEX_POINT('',#227952);
#43620=VERTEX_POINT('',#227954);
#43621=VERTEX_POINT('',#227956);
#43622=VERTEX_POINT('',#227958);
#43623=VERTEX_POINT('',#227960);
#43624=VERTEX_POINT('',#227962);
#43625=VERTEX_POINT('',#227964);
#43626=VERTEX_POINT('',#227966);
#43627=VERTEX_POINT('',#227968);
#43628=VERTEX_POINT('',#227970);
#43629=VERTEX_POINT('',#227977);
#43630=VERTEX_POINT('',#227978);
#43631=VERTEX_POINT('',#227980);
#43632=VERTEX_POINT('',#227982);
#43633=VERTEX_POINT('',#227984);
#43634=VERTEX_POINT('',#227986);
#43635=VERTEX_POINT('',#227988);
#43636=VERTEX_POINT('',#227990);
#43637=VERTEX_POINT('',#227992);
#43638=VERTEX_POINT('',#227994);
#43639=VERTEX_POINT('',#227996);
#43640=VERTEX_POINT('',#227998);
#43641=VERTEX_POINT('',#228002);
#43642=VERTEX_POINT('',#228003);
#43643=VERTEX_POINT('',#228005);
#43644=VERTEX_POINT('',#228007);
#43645=VERTEX_POINT('',#228009);
#43646=VERTEX_POINT('',#228011);
#43647=VERTEX_POINT('',#228013);
#43648=VERTEX_POINT('',#228015);
#43649=VERTEX_POINT('',#228017);
#43650=VERTEX_POINT('',#228019);
#43651=VERTEX_POINT('',#228021);
#43652=VERTEX_POINT('',#228023);
#43653=VERTEX_POINT('',#228027);
#43654=VERTEX_POINT('',#228028);
#43655=VERTEX_POINT('',#228030);
#43656=VERTEX_POINT('',#228032);
#43657=VERTEX_POINT('',#228036);
#43658=VERTEX_POINT('',#228037);
#43659=VERTEX_POINT('',#228039);
#43660=VERTEX_POINT('',#228041);
#43661=VERTEX_POINT('',#228043);
#43662=VERTEX_POINT('',#228045);
#43663=VERTEX_POINT('',#228047);
#43664=VERTEX_POINT('',#228049);
#43665=VERTEX_POINT('',#228051);
#43666=VERTEX_POINT('',#228053);
#43667=VERTEX_POINT('',#228055);
#43668=VERTEX_POINT('',#228057);
#43669=VERTEX_POINT('',#228061);
#43670=VERTEX_POINT('',#228062);
#43671=VERTEX_POINT('',#228064);
#43672=VERTEX_POINT('',#228066);
#43673=VERTEX_POINT('',#228068);
#43674=VERTEX_POINT('',#228070);
#43675=VERTEX_POINT('',#228072);
#43676=VERTEX_POINT('',#228074);
#43677=VERTEX_POINT('',#228076);
#43678=VERTEX_POINT('',#228078);
#43679=VERTEX_POINT('',#228080);
#43680=VERTEX_POINT('',#228082);
#43681=VERTEX_POINT('',#228086);
#43682=VERTEX_POINT('',#228087);
#43683=VERTEX_POINT('',#228089);
#43684=VERTEX_POINT('',#228091);
#43685=VERTEX_POINT('',#228095);
#43686=VERTEX_POINT('',#228096);
#43687=VERTEX_POINT('',#228098);
#43688=VERTEX_POINT('',#228100);
#43689=VERTEX_POINT('',#228102);
#43690=VERTEX_POINT('',#228104);
#43691=VERTEX_POINT('',#228106);
#43692=VERTEX_POINT('',#228108);
#43693=VERTEX_POINT('',#228110);
#43694=VERTEX_POINT('',#228112);
#43695=VERTEX_POINT('',#228114);
#43696=VERTEX_POINT('',#228116);
#43697=VERTEX_POINT('',#228120);
#43698=VERTEX_POINT('',#228121);
#43699=VERTEX_POINT('',#228123);
#43700=VERTEX_POINT('',#228125);
#43701=VERTEX_POINT('',#228127);
#43702=VERTEX_POINT('',#228129);
#43703=VERTEX_POINT('',#228131);
#43704=VERTEX_POINT('',#228133);
#43705=VERTEX_POINT('',#228135);
#43706=VERTEX_POINT('',#228137);
#43707=VERTEX_POINT('',#228139);
#43708=VERTEX_POINT('',#228141);
#43709=VERTEX_POINT('',#228145);
#43710=VERTEX_POINT('',#228146);
#43711=VERTEX_POINT('',#228148);
#43712=VERTEX_POINT('',#228150);
#43713=VERTEX_POINT('',#228154);
#43714=VERTEX_POINT('',#228155);
#43715=VERTEX_POINT('',#228157);
#43716=VERTEX_POINT('',#228159);
#43717=VERTEX_POINT('',#228161);
#43718=VERTEX_POINT('',#228163);
#43719=VERTEX_POINT('',#228165);
#43720=VERTEX_POINT('',#228167);
#43721=VERTEX_POINT('',#228169);
#43722=VERTEX_POINT('',#228171);
#43723=VERTEX_POINT('',#228173);
#43724=VERTEX_POINT('',#228175);
#43725=VERTEX_POINT('',#228179);
#43726=VERTEX_POINT('',#228180);
#43727=VERTEX_POINT('',#228182);
#43728=VERTEX_POINT('',#228184);
#43729=VERTEX_POINT('',#228186);
#43730=VERTEX_POINT('',#228188);
#43731=VERTEX_POINT('',#228190);
#43732=VERTEX_POINT('',#228192);
#43733=VERTEX_POINT('',#228194);
#43734=VERTEX_POINT('',#228196);
#43735=VERTEX_POINT('',#228198);
#43736=VERTEX_POINT('',#228200);
#43737=VERTEX_POINT('',#228204);
#43738=VERTEX_POINT('',#228205);
#43739=VERTEX_POINT('',#228207);
#43740=VERTEX_POINT('',#228209);
#43741=VERTEX_POINT('',#228213);
#43742=VERTEX_POINT('',#228214);
#43743=VERTEX_POINT('',#228216);
#43744=VERTEX_POINT('',#228218);
#43745=VERTEX_POINT('',#228220);
#43746=VERTEX_POINT('',#228222);
#43747=VERTEX_POINT('',#228224);
#43748=VERTEX_POINT('',#228226);
#43749=VERTEX_POINT('',#228228);
#43750=VERTEX_POINT('',#228230);
#43751=VERTEX_POINT('',#228232);
#43752=VERTEX_POINT('',#228234);
#43753=VERTEX_POINT('',#228238);
#43754=VERTEX_POINT('',#228239);
#43755=VERTEX_POINT('',#228241);
#43756=VERTEX_POINT('',#228243);
#43757=VERTEX_POINT('',#228245);
#43758=VERTEX_POINT('',#228247);
#43759=VERTEX_POINT('',#228249);
#43760=VERTEX_POINT('',#228251);
#43761=VERTEX_POINT('',#228253);
#43762=VERTEX_POINT('',#228255);
#43763=VERTEX_POINT('',#228257);
#43764=VERTEX_POINT('',#228259);
#43765=VERTEX_POINT('',#228263);
#43766=VERTEX_POINT('',#228264);
#43767=VERTEX_POINT('',#228266);
#43768=VERTEX_POINT('',#228268);
#43769=VERTEX_POINT('',#228272);
#43770=VERTEX_POINT('',#228273);
#43771=VERTEX_POINT('',#228275);
#43772=VERTEX_POINT('',#228277);
#43773=VERTEX_POINT('',#228279);
#43774=VERTEX_POINT('',#228281);
#43775=VERTEX_POINT('',#228283);
#43776=VERTEX_POINT('',#228285);
#43777=VERTEX_POINT('',#228287);
#43778=VERTEX_POINT('',#228289);
#43779=VERTEX_POINT('',#228291);
#43780=VERTEX_POINT('',#228293);
#43781=VERTEX_POINT('',#228297);
#43782=VERTEX_POINT('',#228298);
#43783=VERTEX_POINT('',#228300);
#43784=VERTEX_POINT('',#228302);
#43785=VERTEX_POINT('',#228304);
#43786=VERTEX_POINT('',#228306);
#43787=VERTEX_POINT('',#228308);
#43788=VERTEX_POINT('',#228310);
#43789=VERTEX_POINT('',#228312);
#43790=VERTEX_POINT('',#228314);
#43791=VERTEX_POINT('',#228316);
#43792=VERTEX_POINT('',#228318);
#43793=VERTEX_POINT('',#228322);
#43794=VERTEX_POINT('',#228323);
#43795=VERTEX_POINT('',#228325);
#43796=VERTEX_POINT('',#228327);
#43797=VERTEX_POINT('',#228331);
#43798=VERTEX_POINT('',#228332);
#43799=VERTEX_POINT('',#228334);
#43800=VERTEX_POINT('',#228336);
#43801=VERTEX_POINT('',#228338);
#43802=VERTEX_POINT('',#228340);
#43803=VERTEX_POINT('',#228342);
#43804=VERTEX_POINT('',#228344);
#43805=VERTEX_POINT('',#228346);
#43806=VERTEX_POINT('',#228348);
#43807=VERTEX_POINT('',#228350);
#43808=VERTEX_POINT('',#228352);
#43809=VERTEX_POINT('',#228356);
#43810=VERTEX_POINT('',#228357);
#43811=VERTEX_POINT('',#228359);
#43812=VERTEX_POINT('',#228361);
#43813=VERTEX_POINT('',#228363);
#43814=VERTEX_POINT('',#228365);
#43815=VERTEX_POINT('',#228367);
#43816=VERTEX_POINT('',#228369);
#43817=VERTEX_POINT('',#228371);
#43818=VERTEX_POINT('',#228373);
#43819=VERTEX_POINT('',#228375);
#43820=VERTEX_POINT('',#228377);
#43821=VERTEX_POINT('',#228381);
#43822=VERTEX_POINT('',#228382);
#43823=VERTEX_POINT('',#228384);
#43824=VERTEX_POINT('',#228386);
#43825=VERTEX_POINT('',#228390);
#43826=VERTEX_POINT('',#228391);
#43827=VERTEX_POINT('',#228393);
#43828=VERTEX_POINT('',#228395);
#43829=VERTEX_POINT('',#228397);
#43830=VERTEX_POINT('',#228399);
#43831=VERTEX_POINT('',#228401);
#43832=VERTEX_POINT('',#228403);
#43833=VERTEX_POINT('',#228405);
#43834=VERTEX_POINT('',#228407);
#43835=VERTEX_POINT('',#228409);
#43836=VERTEX_POINT('',#228411);
#43837=VERTEX_POINT('',#228415);
#43838=VERTEX_POINT('',#228416);
#43839=VERTEX_POINT('',#228418);
#43840=VERTEX_POINT('',#228420);
#43841=VERTEX_POINT('',#228422);
#43842=VERTEX_POINT('',#228424);
#43843=VERTEX_POINT('',#228426);
#43844=VERTEX_POINT('',#228428);
#43845=VERTEX_POINT('',#228430);
#43846=VERTEX_POINT('',#228432);
#43847=VERTEX_POINT('',#228434);
#43848=VERTEX_POINT('',#228436);
#43849=VERTEX_POINT('',#228440);
#43850=VERTEX_POINT('',#228441);
#43851=VERTEX_POINT('',#228443);
#43852=VERTEX_POINT('',#228445);
#43853=VERTEX_POINT('',#228449);
#43854=VERTEX_POINT('',#228450);
#43855=VERTEX_POINT('',#228452);
#43856=VERTEX_POINT('',#228454);
#43857=VERTEX_POINT('',#228456);
#43858=VERTEX_POINT('',#228458);
#43859=VERTEX_POINT('',#228460);
#43860=VERTEX_POINT('',#228462);
#43861=VERTEX_POINT('',#228464);
#43862=VERTEX_POINT('',#228466);
#43863=VERTEX_POINT('',#228468);
#43864=VERTEX_POINT('',#228470);
#43865=VERTEX_POINT('',#228474);
#43866=VERTEX_POINT('',#228475);
#43867=VERTEX_POINT('',#228477);
#43868=VERTEX_POINT('',#228479);
#43869=VERTEX_POINT('',#228481);
#43870=VERTEX_POINT('',#228483);
#43871=VERTEX_POINT('',#228485);
#43872=VERTEX_POINT('',#228487);
#43873=VERTEX_POINT('',#228489);
#43874=VERTEX_POINT('',#228491);
#43875=VERTEX_POINT('',#228493);
#43876=VERTEX_POINT('',#228495);
#43877=VERTEX_POINT('',#228499);
#43878=VERTEX_POINT('',#228500);
#43879=VERTEX_POINT('',#228502);
#43880=VERTEX_POINT('',#228504);
#43881=VERTEX_POINT('',#228508);
#43882=VERTEX_POINT('',#228509);
#43883=VERTEX_POINT('',#228511);
#43884=VERTEX_POINT('',#228513);
#43885=VERTEX_POINT('',#228515);
#43886=VERTEX_POINT('',#228517);
#43887=VERTEX_POINT('',#228519);
#43888=VERTEX_POINT('',#228521);
#43889=VERTEX_POINT('',#228523);
#43890=VERTEX_POINT('',#228525);
#43891=VERTEX_POINT('',#228527);
#43892=VERTEX_POINT('',#228529);
#43893=VERTEX_POINT('',#228533);
#43894=VERTEX_POINT('',#228534);
#43895=VERTEX_POINT('',#228536);
#43896=VERTEX_POINT('',#228538);
#43897=VERTEX_POINT('',#228540);
#43898=VERTEX_POINT('',#228542);
#43899=VERTEX_POINT('',#228544);
#43900=VERTEX_POINT('',#228546);
#43901=VERTEX_POINT('',#228548);
#43902=VERTEX_POINT('',#228550);
#43903=VERTEX_POINT('',#228552);
#43904=VERTEX_POINT('',#228554);
#43905=VERTEX_POINT('',#228558);
#43906=VERTEX_POINT('',#228559);
#43907=VERTEX_POINT('',#228561);
#43908=VERTEX_POINT('',#228563);
#43909=VERTEX_POINT('',#228567);
#43910=VERTEX_POINT('',#228568);
#43911=VERTEX_POINT('',#228570);
#43912=VERTEX_POINT('',#228572);
#43913=VERTEX_POINT('',#228574);
#43914=VERTEX_POINT('',#228576);
#43915=VERTEX_POINT('',#228578);
#43916=VERTEX_POINT('',#228580);
#43917=VERTEX_POINT('',#228582);
#43918=VERTEX_POINT('',#228584);
#43919=VERTEX_POINT('',#228586);
#43920=VERTEX_POINT('',#228588);
#43921=VERTEX_POINT('',#228592);
#43922=VERTEX_POINT('',#228593);
#43923=VERTEX_POINT('',#228595);
#43924=VERTEX_POINT('',#228597);
#43925=VERTEX_POINT('',#228599);
#43926=VERTEX_POINT('',#228601);
#43927=VERTEX_POINT('',#228603);
#43928=VERTEX_POINT('',#228605);
#43929=VERTEX_POINT('',#228607);
#43930=VERTEX_POINT('',#228609);
#43931=VERTEX_POINT('',#228611);
#43932=VERTEX_POINT('',#228613);
#43933=VERTEX_POINT('',#228617);
#43934=VERTEX_POINT('',#228618);
#43935=VERTEX_POINT('',#228620);
#43936=VERTEX_POINT('',#228622);
#43937=VERTEX_POINT('',#228626);
#43938=VERTEX_POINT('',#228627);
#43939=VERTEX_POINT('',#228629);
#43940=VERTEX_POINT('',#228631);
#43941=VERTEX_POINT('',#228633);
#43942=VERTEX_POINT('',#228635);
#43943=VERTEX_POINT('',#228637);
#43944=VERTEX_POINT('',#228639);
#43945=VERTEX_POINT('',#228641);
#43946=VERTEX_POINT('',#228643);
#43947=VERTEX_POINT('',#228645);
#43948=VERTEX_POINT('',#228647);
#43949=VERTEX_POINT('',#228651);
#43950=VERTEX_POINT('',#228652);
#43951=VERTEX_POINT('',#228654);
#43952=VERTEX_POINT('',#228656);
#43953=VERTEX_POINT('',#228658);
#43954=VERTEX_POINT('',#228660);
#43955=VERTEX_POINT('',#228662);
#43956=VERTEX_POINT('',#228664);
#43957=VERTEX_POINT('',#228666);
#43958=VERTEX_POINT('',#228668);
#43959=VERTEX_POINT('',#228670);
#43960=VERTEX_POINT('',#228672);
#43961=VERTEX_POINT('',#228676);
#43962=VERTEX_POINT('',#228677);
#43963=VERTEX_POINT('',#228679);
#43964=VERTEX_POINT('',#228681);
#43965=VERTEX_POINT('',#228685);
#43966=VERTEX_POINT('',#228686);
#43967=VERTEX_POINT('',#228688);
#43968=VERTEX_POINT('',#228690);
#43969=VERTEX_POINT('',#228692);
#43970=VERTEX_POINT('',#228694);
#43971=VERTEX_POINT('',#228696);
#43972=VERTEX_POINT('',#228698);
#43973=VERTEX_POINT('',#228700);
#43974=VERTEX_POINT('',#228702);
#43975=VERTEX_POINT('',#228704);
#43976=VERTEX_POINT('',#228706);
#43977=VERTEX_POINT('',#228710);
#43978=VERTEX_POINT('',#228711);
#43979=VERTEX_POINT('',#228713);
#43980=VERTEX_POINT('',#228715);
#43981=VERTEX_POINT('',#228717);
#43982=VERTEX_POINT('',#228719);
#43983=VERTEX_POINT('',#228721);
#43984=VERTEX_POINT('',#228723);
#43985=VERTEX_POINT('',#228725);
#43986=VERTEX_POINT('',#228727);
#43987=VERTEX_POINT('',#228729);
#43988=VERTEX_POINT('',#228731);
#43989=VERTEX_POINT('',#228735);
#43990=VERTEX_POINT('',#228736);
#43991=VERTEX_POINT('',#228738);
#43992=VERTEX_POINT('',#228740);
#43993=VERTEX_POINT('',#228744);
#43994=VERTEX_POINT('',#228745);
#43995=VERTEX_POINT('',#228747);
#43996=VERTEX_POINT('',#228749);
#43997=VERTEX_POINT('',#228751);
#43998=VERTEX_POINT('',#228753);
#43999=VERTEX_POINT('',#228755);
#44000=VERTEX_POINT('',#228757);
#44001=VERTEX_POINT('',#228759);
#44002=VERTEX_POINT('',#228761);
#44003=VERTEX_POINT('',#228763);
#44004=VERTEX_POINT('',#228765);
#44005=VERTEX_POINT('',#228769);
#44006=VERTEX_POINT('',#228770);
#44007=VERTEX_POINT('',#228772);
#44008=VERTEX_POINT('',#228774);
#44009=VERTEX_POINT('',#228776);
#44010=VERTEX_POINT('',#228778);
#44011=VERTEX_POINT('',#228780);
#44012=VERTEX_POINT('',#228782);
#44013=VERTEX_POINT('',#228784);
#44014=VERTEX_POINT('',#228786);
#44015=VERTEX_POINT('',#228788);
#44016=VERTEX_POINT('',#228790);
#44017=VERTEX_POINT('',#228794);
#44018=VERTEX_POINT('',#228795);
#44019=VERTEX_POINT('',#228797);
#44020=VERTEX_POINT('',#228799);
#44021=VERTEX_POINT('',#228803);
#44022=VERTEX_POINT('',#228804);
#44023=VERTEX_POINT('',#228806);
#44024=VERTEX_POINT('',#228808);
#44025=VERTEX_POINT('',#228810);
#44026=VERTEX_POINT('',#228812);
#44027=VERTEX_POINT('',#228814);
#44028=VERTEX_POINT('',#228816);
#44029=VERTEX_POINT('',#228818);
#44030=VERTEX_POINT('',#228820);
#44031=VERTEX_POINT('',#228822);
#44032=VERTEX_POINT('',#228824);
#44033=VERTEX_POINT('',#228828);
#44034=VERTEX_POINT('',#228829);
#44035=VERTEX_POINT('',#228831);
#44036=VERTEX_POINT('',#228833);
#44037=VERTEX_POINT('',#228835);
#44038=VERTEX_POINT('',#228837);
#44039=VERTEX_POINT('',#228839);
#44040=VERTEX_POINT('',#228841);
#44041=VERTEX_POINT('',#228843);
#44042=VERTEX_POINT('',#228845);
#44043=VERTEX_POINT('',#228847);
#44044=VERTEX_POINT('',#228849);
#44045=VERTEX_POINT('',#253385);
#44046=VERTEX_POINT('',#253387);
#44047=VERTEX_POINT('',#253391);
#44048=VERTEX_POINT('',#253393);
#44049=VERTEX_POINT('',#253397);
#44050=VERTEX_POINT('',#253399);
#44051=VERTEX_POINT('',#253401);
#44052=VERTEX_POINT('',#253405);
#44053=VERTEX_POINT('',#253411);
#44054=VERTEX_POINT('',#253413);
#44055=VERTEX_POINT('',#253420);
#44056=VERTEX_POINT('',#253422);
#44057=VERTEX_POINT('',#253426);
#44058=VERTEX_POINT('',#253428);
#44059=VERTEX_POINT('',#253432);
#44060=VERTEX_POINT('',#253436);
#44061=VERTEX_POINT('',#253442);
#44062=VERTEX_POINT('',#253444);
#44063=VERTEX_POINT('',#253448);
#44064=VERTEX_POINT('',#253449);
#44065=VERTEX_POINT('',#253451);
#44066=VERTEX_POINT('',#253453);
#44067=VERTEX_POINT('',#253457);
#44068=VERTEX_POINT('',#253458);
#44069=VERTEX_POINT('',#253460);
#44070=VERTEX_POINT('',#253462);
#44071=VERTEX_POINT('',#253466);
#44072=VERTEX_POINT('',#253467);
#44073=VERTEX_POINT('',#253469);
#44074=VERTEX_POINT('',#253471);
#44075=VERTEX_POINT('',#253483);
#44076=VERTEX_POINT('',#253484);
#44077=VERTEX_POINT('',#253486);
#44078=VERTEX_POINT('',#253488);
#44079=VERTEX_POINT('',#253500);
#44080=VERTEX_POINT('',#253501);
#44081=VERTEX_POINT('',#253503);
#44082=VERTEX_POINT('',#253505);
#44083=VERTEX_POINT('',#253517);
#44084=VERTEX_POINT('',#253518);
#44085=VERTEX_POINT('',#253520);
#44086=VERTEX_POINT('',#253522);
#44087=VERTEX_POINT('',#253526);
#44088=VERTEX_POINT('',#253528);
#44089=VERTEX_POINT('',#253540);
#44090=VERTEX_POINT('',#253542);
#44091=VERTEX_POINT('',#253546);
#44092=VERTEX_POINT('',#253548);
#44093=VERTEX_POINT('',#253550);
#44094=VERTEX_POINT('',#253555);
#44095=VERTEX_POINT('',#253580);
#44096=VERTEX_POINT('',#253582);
#44097=VERTEX_POINT('',#253605);
#44098=VERTEX_POINT('',#253628);
#44099=VERTEX_POINT('',#253632);
#44100=VERTEX_POINT('',#253633);
#44101=VERTEX_POINT('',#253645);
#44102=VERTEX_POINT('',#253647);
#44103=VERTEX_POINT('',#253651);
#44104=VERTEX_POINT('',#253653);
#44105=VERTEX_POINT('',#253657);
#44106=VERTEX_POINT('',#253659);
#44107=VERTEX_POINT('',#253663);
#44108=VERTEX_POINT('',#253665);
#44109=VERTEX_POINT('',#253669);
#44110=VERTEX_POINT('',#253671);
#44111=VERTEX_POINT('',#253675);
#44112=VERTEX_POINT('',#253677);
#44113=VERTEX_POINT('',#253681);
#44114=VERTEX_POINT('',#253692);
#44115=VERTEX_POINT('',#253694);
#44116=VERTEX_POINT('',#253699);
#44117=VERTEX_POINT('',#253755);
#44118=VERTEX_POINT('',#253757);
#44119=VERTEX_POINT('',#253811);
#44120=VERTEX_POINT('',#253816);
#44121=VERTEX_POINT('',#253872);
#44122=VERTEX_POINT('',#253874);
#44123=VERTEX_POINT('',#253924);
#44124=VERTEX_POINT('',#253929);
#44125=VERTEX_POINT('',#253931);
#44126=VERTEX_POINT('',#253936);
#44127=VERTEX_POINT('',#253992);
#44128=VERTEX_POINT('',#253994);
#44129=VERTEX_POINT('',#254044);
#44130=VERTEX_POINT('',#254049);
#44131=VERTEX_POINT('',#254051);
#44132=VERTEX_POINT('',#254056);
#44133=VERTEX_POINT('',#254106);
#44134=VERTEX_POINT('',#254108);
#44135=VERTEX_POINT('',#254158);
#44136=VERTEX_POINT('',#254163);
#44137=VERTEX_POINT('',#254176);
#44138=VERTEX_POINT('',#254177);
#44139=VERTEX_POINT('',#254179);
#44140=VERTEX_POINT('',#254181);
#44141=VERTEX_POINT('',#254183);
#44142=VERTEX_POINT('',#254190);
#44143=VERTEX_POINT('',#254192);
#44144=VERTEX_POINT('',#254194);
#44145=VERTEX_POINT('',#254196);
#44146=VERTEX_POINT('',#254249);
#44147=VERTEX_POINT('',#254253);
#44148=VERTEX_POINT('',#254254);
#44149=VERTEX_POINT('',#254256);
#44150=VERTEX_POINT('',#254258);
#44151=VERTEX_POINT('',#254260);
#44152=VERTEX_POINT('',#254319);
#44153=VERTEX_POINT('',#254321);
#44154=VERTEX_POINT('',#254323);
#44155=VERTEX_POINT('',#254325);
#44156=VERTEX_POINT('',#254378);
#44157=VERTEX_POINT('',#254382);
#44158=VERTEX_POINT('',#254383);
#44159=VERTEX_POINT('',#254391);
#44160=VERTEX_POINT('',#254392);
#44161=VERTEX_POINT('',#254394);
#44162=VERTEX_POINT('',#254396);
#44163=VERTEX_POINT('',#254400);
#44164=VERTEX_POINT('',#254402);
#44165=VERTEX_POINT('',#254404);
#44166=VERTEX_POINT('',#254465);
#44167=VERTEX_POINT('',#254520);
#44168=VERTEX_POINT('',#254522);
#44169=VERTEX_POINT('',#254524);
#44170=VERTEX_POINT('',#254584);
#44171=VERTEX_POINT('',#254586);
#44172=VERTEX_POINT('',#254588);
#44173=VERTEX_POINT('',#254597);
#44174=VERTEX_POINT('',#254598);
#44175=VERTEX_POINT('',#254661);
#44176=VERTEX_POINT('',#254662);
#44177=VERTEX_POINT('',#254664);
#44178=VERTEX_POINT('',#254666);
#44179=VERTEX_POINT('',#254670);
#44180=VERTEX_POINT('',#254672);
#44181=VERTEX_POINT('',#254676);
#44182=VERTEX_POINT('',#254678);
#44183=VERTEX_POINT('',#254682);
#44184=VERTEX_POINT('',#254684);
#44185=VERTEX_POINT('',#254688);
#44186=VERTEX_POINT('',#254690);
#44187=VERTEX_POINT('',#254694);
#44188=VERTEX_POINT('',#254696);
#44189=VERTEX_POINT('',#254700);
#44190=VERTEX_POINT('',#254702);
#44191=VERTEX_POINT('',#254709);
#44192=VERTEX_POINT('',#254756);
#44193=VERTEX_POINT('',#254758);
#44194=VERTEX_POINT('',#254760);
#44195=VERTEX_POINT('',#254809);
#44196=VERTEX_POINT('',#254810);
#44197=VERTEX_POINT('',#254815);
#44198=VERTEX_POINT('',#254817);
#44199=VERTEX_POINT('',#254819);
#44200=VERTEX_POINT('',#254830);
#44201=VERTEX_POINT('',#254838);
#44202=VERTEX_POINT('',#254845);
#44203=VERTEX_POINT('',#254849);
#44204=VERTEX_POINT('',#254850);
#44205=VERTEX_POINT('',#254852);
#44206=VERTEX_POINT('',#254854);
#44207=VERTEX_POINT('',#254859);
#44208=VERTEX_POINT('',#254861);
#44209=VERTEX_POINT('',#254863);
#44210=VERTEX_POINT('',#254870);
#44211=VERTEX_POINT('',#254963);
#44212=VERTEX_POINT('',#254970);
#44213=VERTEX_POINT('',#254994);
#44214=VERTEX_POINT('',#254995);
#44215=VERTEX_POINT('',#254997);
#44216=VERTEX_POINT('',#254999);
#44217=VERTEX_POINT('',#255003);
#44218=VERTEX_POINT('',#255005);
#44219=VERTEX_POINT('',#255023);
#44220=VERTEX_POINT('',#255027);
#44221=VERTEX_POINT('',#255028);
#44222=VERTEX_POINT('',#255030);
#44223=VERTEX_POINT('',#255045);
#44224=VERTEX_POINT('',#255047);
#44225=VERTEX_POINT('',#255051);
#44226=VERTEX_POINT('',#255052);
#44227=VERTEX_POINT('',#255057);
#44228=VERTEX_POINT('',#255058);
#44229=VERTEX_POINT('',#255060);
#44230=VERTEX_POINT('',#255062);
#44231=VERTEX_POINT('',#255068);
#44232=VERTEX_POINT('',#255069);
#44233=VERTEX_POINT('',#255071);
#44234=VERTEX_POINT('',#255073);
#44235=VERTEX_POINT('',#255077);
#44236=VERTEX_POINT('',#255078);
#44237=VERTEX_POINT('',#255080);
#44238=VERTEX_POINT('',#255082);
#44239=VERTEX_POINT('',#255086);
#44240=VERTEX_POINT('',#255088);
#44241=VERTEX_POINT('',#255092);
#44242=VERTEX_POINT('',#255094);
#44243=VERTEX_POINT('',#255098);
#44244=VERTEX_POINT('',#255100);
#44245=VERTEX_POINT('',#255153);
#44246=VERTEX_POINT('',#255163);
#44247=VERTEX_POINT('',#255165);
#44248=VERTEX_POINT('',#255173);
#44249=VERTEX_POINT('',#255225);
#44250=VERTEX_POINT('',#255278);
#44251=VERTEX_POINT('',#255289);
#44252=VERTEX_POINT('',#255290);
#44253=VERTEX_POINT('',#255292);
#44254=VERTEX_POINT('',#255294);
#44255=VERTEX_POINT('',#255300);
#44256=VERTEX_POINT('',#255302);
#44257=VERTEX_POINT('',#255361);
#44258=VERTEX_POINT('',#255362);
#44259=VERTEX_POINT('',#255364);
#44260=VERTEX_POINT('',#255417);
#44261=VERTEX_POINT('',#255428);
#44262=VERTEX_POINT('',#255429);
#44263=VERTEX_POINT('',#255431);
#44264=VERTEX_POINT('',#255433);
#44265=VERTEX_POINT('',#255435);
#44266=VERTEX_POINT('',#255437);
#44267=VERTEX_POINT('',#255439);
#44268=VERTEX_POINT('',#255441);
#44269=VERTEX_POINT('',#255445);
#44270=VERTEX_POINT('',#255447);
#44271=VERTEX_POINT('',#255455);
#44272=VERTEX_POINT('',#255505);
#44273=VERTEX_POINT('',#255509);
#44274=VERTEX_POINT('',#255511);
#44275=VERTEX_POINT('',#255564);
#44276=VERTEX_POINT('',#255575);
#44277=VERTEX_POINT('',#255576);
#44278=VERTEX_POINT('',#255578);
#44279=VERTEX_POINT('',#255580);
#44280=VERTEX_POINT('',#255585);
#44281=VERTEX_POINT('',#255587);
#44282=VERTEX_POINT('',#255625);
#44283=VERTEX_POINT('',#255707);
#44284=VERTEX_POINT('',#255720);
#44285=VERTEX_POINT('',#255802);
#44286=VERTEX_POINT('',#255815);
#44287=VERTEX_POINT('',#255896);
#44288=VERTEX_POINT('',#255909);
#44289=VERTEX_POINT('',#255920);
#44290=VERTEX_POINT('',#255954);
#44291=VERTEX_POINT('',#255967);
#44292=VERTEX_POINT('',#256048);
#44293=VERTEX_POINT('',#256061);
#44294=VERTEX_POINT('',#256142);
#44295=VERTEX_POINT('',#256166);
#44296=VERTEX_POINT('',#256190);
#44297=VERTEX_POINT('',#257718);
#44298=VERTEX_POINT('',#257952);
#44299=VERTEX_POINT('',#258186);
#44300=VERTEX_POINT('',#258420);
#44301=VERTEX_POINT('',#258654);
#44302=VERTEX_POINT('',#258882);
#44303=VERTEX_POINT('',#258896);
#44304=VERTEX_POINT('',#259067);
#44305=VERTEX_POINT('',#259304);
#44306=VERTEX_POINT('',#260910);
#44307=VERTEX_POINT('',#260911);
#44308=VERTEX_POINT('',#260914);
#44309=VERTEX_POINT('',#260915);
#44310=VERTEX_POINT('',#260917);
#44311=VERTEX_POINT('',#260922);
#44312=VERTEX_POINT('',#260923);
#44313=VERTEX_POINT('',#260925);
#44314=VERTEX_POINT('',#260995);
#44315=VERTEX_POINT('',#260996);
#44316=VERTEX_POINT('',#261223);
#44317=VERTEX_POINT('',#261225);
#44318=VERTEX_POINT('',#261263);
#44319=VERTEX_POINT('',#261265);
#44320=VERTEX_POINT('',#261274);
#44321=VERTEX_POINT('',#261325);
#44322=VERTEX_POINT('',#261327);
#44323=VERTEX_POINT('',#261413);
#44324=VERTEX_POINT('',#261477);
#44325=VERTEX_POINT('',#261478);
#44326=VERTEX_POINT('',#261480);
#44327=VERTEX_POINT('',#261485);
#44328=VERTEX_POINT('',#261487);
#44329=VERTEX_POINT('',#261489);
#44330=VERTEX_POINT('',#261493);
#44331=VERTEX_POINT('',#261528);
#44332=VERTEX_POINT('',#261530);
#44333=VERTEX_POINT('',#261569);
#44334=VERTEX_POINT('',#261573);
#44335=VERTEX_POINT('',#261579);
#44336=VERTEX_POINT('',#261581);
#44337=VERTEX_POINT('',#261585);
#44338=VERTEX_POINT('',#261587);
#44339=VERTEX_POINT('',#261589);
#44340=VERTEX_POINT('',#261593);
#44341=VERTEX_POINT('',#261594);
#44342=VERTEX_POINT('',#261597);
#44343=VERTEX_POINT('',#261601);
#44344=VERTEX_POINT('',#261603);
#44345=VERTEX_POINT('',#261607);
#44346=VERTEX_POINT('',#261609);
#44347=VERTEX_POINT('',#261613);
#44348=VERTEX_POINT('',#261615);
#44349=VERTEX_POINT('',#261623);
#44350=VERTEX_POINT('',#261627);
#44351=VERTEX_POINT('',#261631);
#44352=VERTEX_POINT('',#261633);
#44353=VERTEX_POINT('',#261642);
#44354=VERTEX_POINT('',#261643);
#44355=VERTEX_POINT('',#261645);
#44356=VERTEX_POINT('',#261661);
#44357=VERTEX_POINT('',#261679);
#44358=VERTEX_POINT('',#261680);
#44359=VERTEX_POINT('',#261717);
#44360=VERTEX_POINT('',#261718);
#44361=VERTEX_POINT('',#261755);
#44362=VERTEX_POINT('',#261756);
#44363=VERTEX_POINT('',#261793);
#44364=VERTEX_POINT('',#261794);
#44365=VERTEX_POINT('',#261831);
#44366=VERTEX_POINT('',#261832);
#44367=VERTEX_POINT('',#261869);
#44368=VERTEX_POINT('',#261870);
#44369=VERTEX_POINT('',#261872);
#44370=VERTEX_POINT('',#261885);
#44371=VERTEX_POINT('',#261886);
#44372=VERTEX_POINT('',#261924);
#44373=VERTEX_POINT('',#261939);
#44374=VERTEX_POINT('',#261940);
#44375=VERTEX_POINT('',#262015);
#44376=VERTEX_POINT('',#262016);
#44377=VERTEX_POINT('',#262091);
#44378=VERTEX_POINT('',#262092);
#44379=VERTEX_POINT('',#262167);
#44380=VERTEX_POINT('',#262168);
#44381=VERTEX_POINT('',#262243);
#44382=VERTEX_POINT('',#262244);
#44383=VERTEX_POINT('',#262321);
#44384=VERTEX_POINT('',#262322);
#44385=VERTEX_POINT('',#262324);
#44386=VERTEX_POINT('',#262387);
#44387=VERTEX_POINT('',#262389);
#44388=VERTEX_POINT('',#262392);
#44389=VERTEX_POINT('',#262396);
#44390=VERTEX_POINT('',#262397);
#44391=VERTEX_POINT('',#262402);
#44392=VERTEX_POINT('',#262428);
#44393=VERTEX_POINT('',#262429);
#44394=VERTEX_POINT('',#262431);
#44395=VERTEX_POINT('',#262433);
#44396=VERTEX_POINT('',#262435);
#44397=VERTEX_POINT('',#262437);
#44398=VERTEX_POINT('',#262465);
#44399=VERTEX_POINT('',#262466);
#44400=VERTEX_POINT('',#262468);
#44401=VERTEX_POINT('',#262470);
#44402=VERTEX_POINT('',#262472);
#44403=VERTEX_POINT('',#262474);
#44404=VERTEX_POINT('',#263169);
#44405=VERTEX_POINT('',#263170);
#44406=VERTEX_POINT('',#263172);
#44407=VERTEX_POINT('',#263188);
#44408=VERTEX_POINT('',#263206);
#44409=VERTEX_POINT('',#263207);
#44410=VERTEX_POINT('',#263244);
#44411=VERTEX_POINT('',#263245);
#44412=VERTEX_POINT('',#263282);
#44413=VERTEX_POINT('',#263283);
#44414=VERTEX_POINT('',#263320);
#44415=VERTEX_POINT('',#263321);
#44416=VERTEX_POINT('',#263358);
#44417=VERTEX_POINT('',#263359);
#44418=VERTEX_POINT('',#263396);
#44419=VERTEX_POINT('',#263397);
#44420=VERTEX_POINT('',#263399);
#44421=VERTEX_POINT('',#263412);
#44422=VERTEX_POINT('',#263413);
#44423=VERTEX_POINT('',#263451);
#44424=VERTEX_POINT('',#263466);
#44425=VERTEX_POINT('',#263467);
#44426=VERTEX_POINT('',#263542);
#44427=VERTEX_POINT('',#263543);
#44428=VERTEX_POINT('',#263618);
#44429=VERTEX_POINT('',#263619);
#44430=VERTEX_POINT('',#263694);
#44431=VERTEX_POINT('',#263695);
#44432=VERTEX_POINT('',#263770);
#44433=VERTEX_POINT('',#263771);
#44434=VERTEX_POINT('',#263848);
#44435=VERTEX_POINT('',#263849);
#44436=VERTEX_POINT('',#263851);
#44437=VERTEX_POINT('',#263914);
#44438=VERTEX_POINT('',#263916);
#44439=VERTEX_POINT('',#263919);
#44440=VERTEX_POINT('',#263923);
#44441=VERTEX_POINT('',#263924);
#44442=VERTEX_POINT('',#263929);
#44443=VERTEX_POINT('',#263955);
#44444=VERTEX_POINT('',#263956);
#44445=VERTEX_POINT('',#263958);
#44446=VERTEX_POINT('',#263960);
#44447=VERTEX_POINT('',#263962);
#44448=VERTEX_POINT('',#263964);
#44449=VERTEX_POINT('',#263992);
#44450=VERTEX_POINT('',#263993);
#44451=VERTEX_POINT('',#263995);
#44452=VERTEX_POINT('',#263997);
#44453=VERTEX_POINT('',#263999);
#44454=VERTEX_POINT('',#264001);
#44455=VERTEX_POINT('',#264696);
#44456=VERTEX_POINT('',#264698);
#44457=VERTEX_POINT('',#264702);
#44458=VERTEX_POINT('',#264703);
#44459=VERTEX_POINT('',#264706);
#44460=VERTEX_POINT('',#264710);
#44461=VERTEX_POINT('',#264712);
#44462=VERTEX_POINT('',#264716);
#44463=VERTEX_POINT('',#264717);
#44464=VERTEX_POINT('',#264720);
#44465=VERTEX_POINT('',#264724);
#44466=VERTEX_POINT('',#264726);
#44467=VERTEX_POINT('',#264765);
#44468=VERTEX_POINT('',#264766);
#44469=VERTEX_POINT('',#264805);
#44470=VERTEX_POINT('',#264842);
#44471=VERTEX_POINT('',#264844);
#44472=VERTEX_POINT('',#264888);
#44473=VERTEX_POINT('',#264890);
#44474=VERTEX_POINT('',#264894);
#44475=VERTEX_POINT('',#264896);
#44476=VERTEX_POINT('',#264900);
#44477=VERTEX_POINT('',#264902);
#44478=VERTEX_POINT('',#264904);
#44479=VERTEX_POINT('',#264908);
#44480=VERTEX_POINT('',#264912);
#44481=VERTEX_POINT('',#264913);
#44482=VERTEX_POINT('',#264915);
#44483=VERTEX_POINT('',#264917);
#44484=VERTEX_POINT('',#264921);
#44485=VERTEX_POINT('',#264923);
#44486=VERTEX_POINT('',#264927);
#44487=VERTEX_POINT('',#264929);
#44488=VERTEX_POINT('',#264933);
#44489=VERTEX_POINT('',#264935);
#44490=VERTEX_POINT('',#264939);
#44491=VERTEX_POINT('',#264941);
#44492=VERTEX_POINT('',#264945);
#44493=VERTEX_POINT('',#264947);
#44494=VERTEX_POINT('',#264951);
#44495=VERTEX_POINT('',#264953);
#44496=VERTEX_POINT('',#264957);
#44497=VERTEX_POINT('',#264959);
#44498=VERTEX_POINT('',#264963);
#44499=VERTEX_POINT('',#264965);
#44500=VERTEX_POINT('',#264969);
#44501=VERTEX_POINT('',#264971);
#44502=VERTEX_POINT('',#264975);
#44503=VERTEX_POINT('',#264977);
#44504=VERTEX_POINT('',#264981);
#44505=VERTEX_POINT('',#264982);
#44506=VERTEX_POINT('',#264984);
#44507=VERTEX_POINT('',#264986);
#44508=VERTEX_POINT('',#264990);
#44509=VERTEX_POINT('',#264992);
#44510=VERTEX_POINT('',#264996);
#44511=VERTEX_POINT('',#264998);
#44512=VERTEX_POINT('',#265002);
#44513=VERTEX_POINT('',#265004);
#44514=VERTEX_POINT('',#265008);
#44515=VERTEX_POINT('',#265010);
#44516=VERTEX_POINT('',#265014);
#44517=VERTEX_POINT('',#265016);
#44518=VERTEX_POINT('',#265020);
#44519=VERTEX_POINT('',#265022);
#44520=VERTEX_POINT('',#265029);
#44521=VERTEX_POINT('',#265030);
#44522=VERTEX_POINT('',#265032);
#44523=VERTEX_POINT('',#265034);
#44524=VERTEX_POINT('',#265036);
#44525=VERTEX_POINT('',#265038);
#44526=VERTEX_POINT('',#265040);
#44527=VERTEX_POINT('',#265042);
#44528=VERTEX_POINT('',#265050);
#44529=VERTEX_POINT('',#265051);
#44530=VERTEX_POINT('',#265053);
#44531=VERTEX_POINT('',#265055);
#44532=VERTEX_POINT('',#265057);
#44533=VERTEX_POINT('',#265059);
#44534=VERTEX_POINT('',#265061);
#44535=VERTEX_POINT('',#265063);
#44536=VERTEX_POINT('',#265067);
#44537=VERTEX_POINT('',#265069);
#44538=VERTEX_POINT('',#265073);
#44539=VERTEX_POINT('',#265077);
#44540=VERTEX_POINT('',#265081);
#44541=VERTEX_POINT('',#265085);
#44542=VERTEX_POINT('',#265089);
#44543=VERTEX_POINT('',#265093);
#44544=VERTEX_POINT('',#265116);
#44545=VERTEX_POINT('',#265117);
#44546=VERTEX_POINT('',#265119);
#44547=VERTEX_POINT('',#265121);
#44548=VERTEX_POINT('',#265125);
#44549=VERTEX_POINT('',#265127);
#44550=VERTEX_POINT('',#265130);
#44551=VERTEX_POINT('',#265132);
#44552=VERTEX_POINT('',#265139);
#44553=VERTEX_POINT('',#265141);
#44554=VERTEX_POINT('',#265149);
#44555=VERTEX_POINT('',#265151);
#45747=EDGE_CURVE('',#36725,#36725,#30456,.T.);
#45748=EDGE_CURVE('',#36725,#36726,#30457,.T.);
#45749=EDGE_CURVE('',#36726,#36727,#30458,.T.);
#45750=EDGE_CURVE('',#36727,#36726,#30459,.T.);
#45751=EDGE_CURVE('',#36728,#36729,#4243,.F.);
#45752=EDGE_CURVE('',#36730,#36728,#20078,.T.);
#45753=EDGE_CURVE('',#36731,#36730,#4244,.F.);
#45754=EDGE_CURVE('',#36729,#36731,#20079,.T.);
#45755=EDGE_CURVE('',#36732,#36733,#30460,.T.);
#45756=EDGE_CURVE('',#36731,#36732,#4085,.T.);
#45757=EDGE_CURVE('',#36733,#36730,#4086,.T.);
#45758=EDGE_CURVE('',#36734,#36734,#30461,.T.);
#45759=EDGE_CURVE('',#36734,#36735,#20080,.T.);
#45760=EDGE_CURVE('',#36735,#36735,#30462,.T.);
#45761=EDGE_CURVE('',#36736,#36737,#30463,.T.);
#45762=EDGE_CURVE('',#36738,#36736,#4087,.T.);
#45763=EDGE_CURVE('',#36738,#36739,#4245,.T.);
#45764=EDGE_CURVE('',#36740,#36739,#4088,.T.);
#45765=EDGE_CURVE('',#36737,#36740,#30464,.T.);
#45766=EDGE_CURVE('',#36741,#36742,#30465,.T.);
#45767=EDGE_CURVE('',#36742,#36743,#30466,.T.);
#45768=EDGE_CURVE('',#36743,#36736,#30467,.T.);
#45769=EDGE_CURVE('',#36737,#36727,#20081,.T.);
#45770=EDGE_CURVE('',#36740,#36744,#30468,.T.);
#45771=EDGE_CURVE('',#36744,#36741,#30469,.T.);
#45772=EDGE_CURVE('',#36745,#36745,#30470,.T.);
#45773=EDGE_CURVE('',#36746,#36747,#30471,.T.);
#45774=EDGE_CURVE('',#36747,#36746,#30472,.T.);
#45775=EDGE_CURVE('',#36747,#36745,#30473,.T.);
#45776=EDGE_CURVE('',#36746,#36748,#20082,.T.);
#45777=EDGE_CURVE('',#36749,#36748,#30474,.T.);
#45778=EDGE_CURVE('',#36748,#36749,#30475,.T.);
#45779=EDGE_CURVE('',#36750,#36750,#30476,.T.);
#45780=EDGE_CURVE('',#36750,#36749,#30477,.T.);
#45781=EDGE_CURVE('',#36751,#36751,#30478,.T.);
#45782=EDGE_CURVE('',#36751,#36752,#20083,.T.);
#45783=EDGE_CURVE('',#36752,#36752,#30479,.T.);
#45784=EDGE_CURVE('',#36728,#36741,#4089,.T.);
#45785=EDGE_CURVE('',#36742,#36729,#4090,.T.);
#45786=EDGE_CURVE('',#36753,#36744,#4091,.T.);
#45787=EDGE_CURVE('',#36753,#36754,#4246,.T.);
#45788=EDGE_CURVE('',#36741,#36754,#4092,.T.);
#45789=EDGE_CURVE('',#36755,#36740,#4093,.T.);
#45790=EDGE_CURVE('',#36755,#36756,#4247,.T.);
#45791=EDGE_CURVE('',#36744,#36756,#4094,.T.);
#45792=EDGE_CURVE('',#36757,#36743,#4095,.T.);
#45793=EDGE_CURVE('',#36757,#36758,#4248,.T.);
#45794=EDGE_CURVE('',#36736,#36758,#4096,.T.);
#45795=EDGE_CURVE('',#36759,#36742,#4097,.T.);
#45796=EDGE_CURVE('',#36759,#36760,#4249,.T.);
#45797=EDGE_CURVE('',#36743,#36760,#4098,.T.);
#45798=EDGE_CURVE('',#36733,#36761,#30480,.T.);
#45799=EDGE_CURVE('',#36761,#36762,#30481,.T.);
#45800=EDGE_CURVE('',#36762,#36763,#30482,.T.);
#45801=EDGE_CURVE('',#36763,#36764,#30483,.T.);
#45802=EDGE_CURVE('',#36764,#36732,#30484,.T.);
#45803=EDGE_CURVE('',#36765,#36764,#4099,.T.);
#45804=EDGE_CURVE('',#36765,#36766,#4250,.T.);
#45805=EDGE_CURVE('',#36732,#36766,#4100,.T.);
#45806=EDGE_CURVE('',#36767,#36763,#4101,.T.);
#45807=EDGE_CURVE('',#36767,#36768,#4251,.T.);
#45808=EDGE_CURVE('',#36764,#36768,#4102,.T.);
#45809=EDGE_CURVE('',#36769,#36762,#4103,.T.);
#45810=EDGE_CURVE('',#36769,#36770,#4252,.T.);
#45811=EDGE_CURVE('',#36763,#36770,#4104,.T.);
#45812=EDGE_CURVE('',#36771,#36761,#4105,.T.);
#45813=EDGE_CURVE('',#36771,#36772,#4253,.T.);
#45814=EDGE_CURVE('',#36762,#36772,#4106,.T.);
#45815=EDGE_CURVE('',#36773,#36733,#4107,.T.);
#45816=EDGE_CURVE('',#36773,#36774,#4254,.T.);
#45817=EDGE_CURVE('',#36761,#36774,#4108,.T.);
#45818=EDGE_CURVE('',#36754,#36773,#20084,.T.);
#45819=EDGE_CURVE('',#36774,#36753,#20085,.T.);
#45820=EDGE_CURVE('',#36756,#36771,#20086,.T.);
#45821=EDGE_CURVE('',#36772,#36755,#20087,.T.);
#45822=EDGE_CURVE('',#36739,#36769,#20088,.T.);
#45823=EDGE_CURVE('',#36758,#36767,#20089,.T.);
#45824=EDGE_CURVE('',#36770,#36738,#20090,.T.);
#45825=EDGE_CURVE('',#36760,#36765,#20091,.T.);
#45826=EDGE_CURVE('',#36768,#36757,#20092,.T.);
#45827=EDGE_CURVE('',#36766,#36759,#20093,.T.);
#45828=EDGE_CURVE('',#36775,#36775,#30485,.T.);
#45829=EDGE_CURVE('',#36775,#36776,#20094,.T.);
#45830=EDGE_CURVE('',#36776,#36776,#30486,.T.);
#45831=EDGE_CURVE('',#36777,#36777,#30487,.T.);
#45832=EDGE_CURVE('',#36777,#36778,#20095,.T.);
#45833=EDGE_CURVE('',#36778,#36778,#30488,.T.);
#45834=EDGE_CURVE('',#36779,#36779,#30489,.T.);
#45835=EDGE_CURVE('',#36779,#36780,#20096,.T.);
#45836=EDGE_CURVE('',#36780,#36780,#30490,.T.);
#45837=EDGE_CURVE('',#36781,#36781,#30491,.T.);
#45838=EDGE_CURVE('',#36781,#36782,#20097,.T.);
#45839=EDGE_CURVE('',#36782,#36782,#30492,.T.);
#45840=EDGE_CURVE('',#36783,#36783,#30493,.T.);
#45841=EDGE_CURVE('',#36783,#36784,#20098,.T.);
#45842=EDGE_CURVE('',#36784,#36784,#30494,.T.);
#45843=EDGE_CURVE('',#36785,#36785,#30495,.T.);
#45844=EDGE_CURVE('',#36785,#36786,#20099,.T.);
#45845=EDGE_CURVE('',#36786,#36786,#30496,.T.);
#45846=EDGE_CURVE('',#36787,#36787,#30497,.T.);
#45847=EDGE_CURVE('',#36787,#36788,#20100,.T.);
#45848=EDGE_CURVE('',#36788,#36788,#30498,.T.);
#45849=EDGE_CURVE('',#36789,#36789,#30499,.T.);
#45850=EDGE_CURVE('',#36789,#36790,#20101,.T.);
#45851=EDGE_CURVE('',#36790,#36790,#30500,.T.);
#45852=EDGE_CURVE('',#36791,#36792,#30501,.T.);
#45853=EDGE_CURVE('',#36792,#36791,#30502,.T.);
#45854=EDGE_CURVE('',#36792,#36793,#30503,.T.);
#45855=EDGE_CURVE('',#36793,#36793,#30504,.T.);
#45856=EDGE_CURVE('',#36794,#36794,#30505,.T.);
#45857=EDGE_CURVE('',#36794,#36795,#30506,.T.);
#45858=EDGE_CURVE('',#36796,#36795,#30507,.T.);
#45859=EDGE_CURVE('',#36795,#36796,#30508,.T.);
#45860=EDGE_CURVE('',#36797,#36797,#30509,.T.);
#45861=EDGE_CURVE('',#36797,#36796,#20102,.T.);
#45862=EDGE_CURVE('',#36791,#36798,#20103,.T.);
#45863=EDGE_CURVE('',#36798,#36798,#30510,.T.);
#45864=EDGE_CURVE('',#36799,#36799,#30511,.T.);
#45865=EDGE_CURVE('',#36799,#36800,#30512,.T.);
#45866=EDGE_CURVE('',#36801,#36800,#30513,.T.);
#45867=EDGE_CURVE('',#36800,#36801,#30514,.T.);
#45868=EDGE_CURVE('',#36802,#36803,#30515,.T.);
#45869=EDGE_CURVE('',#36803,#36802,#30516,.T.);
#45870=EDGE_CURVE('',#36803,#36804,#30517,.T.);
#45871=EDGE_CURVE('',#36804,#36804,#30518,.T.);
#45872=EDGE_CURVE('',#36805,#36805,#30519,.T.);
#45873=EDGE_CURVE('',#36805,#36801,#20104,.T.);
#45874=EDGE_CURVE('',#36802,#36806,#20105,.T.);
#45875=EDGE_CURVE('',#36806,#36806,#30520,.T.);
#45876=EDGE_CURVE('',#36807,#36807,#30521,.T.);
#45877=EDGE_CURVE('',#36807,#36808,#20106,.T.);
#45878=EDGE_CURVE('',#36808,#36808,#30522,.T.);
#45879=EDGE_CURVE('',#36809,#36809,#30523,.T.);
#45880=EDGE_CURVE('',#36809,#36810,#20107,.T.);
#45881=EDGE_CURVE('',#36810,#36810,#30524,.T.);
#45882=EDGE_CURVE('',#36811,#36812,#30525,.T.);
#45883=EDGE_CURVE('',#36813,#36811,#30526,.T.);
#45884=EDGE_CURVE('',#36814,#36813,#30527,.T.);
#45885=EDGE_CURVE('',#36814,#36812,#30528,.T.);
#45886=EDGE_CURVE('',#36815,#36816,#30529,.T.);
#45887=EDGE_CURVE('',#36817,#36815,#30530,.T.);
#45888=EDGE_CURVE('',#36818,#36817,#30531,.T.);
#45889=EDGE_CURVE('',#36818,#36816,#30532,.T.);
#45890=EDGE_CURVE('',#36819,#36820,#30533,.T.);
#45891=EDGE_CURVE('',#36821,#36819,#30534,.T.);
#45892=EDGE_CURVE('',#36822,#36821,#30535,.T.);
#45893=EDGE_CURVE('',#36822,#36820,#30536,.T.);
#45894=EDGE_CURVE('',#36823,#36824,#30537,.T.);
#45895=EDGE_CURVE('',#36825,#36823,#30538,.T.);
#45896=EDGE_CURVE('',#36826,#36825,#30539,.T.);
#45897=EDGE_CURVE('',#36826,#36827,#30540,.T.);
#45898=EDGE_CURVE('',#36824,#36827,#30541,.T.);
#45899=EDGE_CURVE('',#36828,#36828,#30542,.T.);
#45900=EDGE_CURVE('',#36828,#36829,#30543,.T.);
#45901=EDGE_CURVE('',#36830,#36829,#30544,.T.);
#45902=EDGE_CURVE('',#36829,#36830,#30545,.T.);
#45903=EDGE_CURVE('',#36831,#36831,#30546,.T.);
#45904=EDGE_CURVE('',#36831,#36832,#30547,.T.);
#45905=EDGE_CURVE('',#36832,#36832,#30548,.T.);
#45906=EDGE_CURVE('',#36833,#36833,#30549,.T.);
#45907=EDGE_CURVE('',#36833,#36834,#30550,.T.);
#45908=EDGE_CURVE('',#36835,#36834,#30551,.T.);
#45909=EDGE_CURVE('',#36834,#36835,#30552,.T.);
#45910=EDGE_CURVE('',#36836,#36836,#30553,.T.);
#45911=EDGE_CURVE('',#36836,#36837,#30554,.T.);
#45912=EDGE_CURVE('',#36837,#36837,#30555,.T.);
#45913=EDGE_CURVE('',#36838,#36838,#30556,.T.);
#45914=EDGE_CURVE('',#36838,#36839,#20108,.T.);
#45915=EDGE_CURVE('',#36839,#36839,#30557,.T.);
#45916=EDGE_CURVE('',#36839,#36836,#20109,.T.);
#45917=EDGE_CURVE('',#36840,#36841,#30558,.T.);
#45918=EDGE_CURVE('',#36841,#36842,#4255,.T.);
#45919=EDGE_CURVE('',#36842,#36843,#20110,.T.);
#45920=EDGE_CURVE('',#36843,#36844,#30559,.T.);
#45921=EDGE_CURVE('',#36844,#36845,#20111,.T.);
#45922=EDGE_CURVE('',#36845,#36846,#4256,.T.);
#45923=EDGE_CURVE('',#36846,#36847,#30560,.T.);
#45924=EDGE_CURVE('',#36847,#36848,#4257,.T.);
#45925=EDGE_CURVE('',#36848,#36849,#20112,.T.);
#45926=EDGE_CURVE('',#36849,#36850,#30561,.T.);
#45927=EDGE_CURVE('',#36850,#36851,#20113,.T.);
#45928=EDGE_CURVE('',#36851,#36852,#4258,.T.);
#45929=EDGE_CURVE('',#36852,#36853,#30562,.T.);
#45930=EDGE_CURVE('',#36853,#36854,#4259,.T.);
#45931=EDGE_CURVE('',#36854,#36855,#20114,.T.);
#45932=EDGE_CURVE('',#36855,#36856,#30563,.T.);
#45933=EDGE_CURVE('',#36856,#36857,#20115,.T.);
#45934=EDGE_CURVE('',#36857,#36858,#4260,.T.);
#45935=EDGE_CURVE('',#36858,#36859,#30564,.T.);
#45936=EDGE_CURVE('',#36859,#36860,#4261,.T.);
#45937=EDGE_CURVE('',#36860,#36861,#20116,.T.);
#45938=EDGE_CURVE('',#36861,#36862,#30565,.T.);
#45939=EDGE_CURVE('',#36862,#36863,#20117,.T.);
#45940=EDGE_CURVE('',#36863,#36864,#4262,.T.);
#45941=EDGE_CURVE('',#36864,#36865,#30566,.T.);
#45942=EDGE_CURVE('',#36865,#36866,#4263,.T.);
#45943=EDGE_CURVE('',#36866,#36867,#20118,.T.);
#45944=EDGE_CURVE('',#36867,#36868,#30567,.T.);
#45945=EDGE_CURVE('',#36868,#36869,#20119,.T.);
#45946=EDGE_CURVE('',#36869,#36870,#4264,.T.);
#45947=EDGE_CURVE('',#36870,#36871,#30568,.T.);
#45948=EDGE_CURVE('',#36871,#36872,#4265,.T.);
#45949=EDGE_CURVE('',#36872,#36873,#20120,.T.);
#45950=EDGE_CURVE('',#36873,#36874,#30569,.T.);
#45951=EDGE_CURVE('',#36874,#36875,#20121,.T.);
#45952=EDGE_CURVE('',#36875,#36876,#4266,.T.);
#45953=EDGE_CURVE('',#36876,#36877,#30570,.T.);
#45954=EDGE_CURVE('',#36877,#36878,#4267,.T.);
#45955=EDGE_CURVE('',#36878,#36879,#20122,.T.);
#45956=EDGE_CURVE('',#36879,#36880,#30571,.T.);
#45957=EDGE_CURVE('',#36880,#36881,#20123,.T.);
#45958=EDGE_CURVE('',#36881,#36882,#4268,.T.);
#45959=EDGE_CURVE('',#36882,#36883,#30572,.T.);
#45960=EDGE_CURVE('',#36883,#36884,#4269,.T.);
#45961=EDGE_CURVE('',#36884,#36885,#20124,.T.);
#45962=EDGE_CURVE('',#36885,#36886,#30573,.T.);
#45963=EDGE_CURVE('',#36886,#36887,#20125,.T.);
#45964=EDGE_CURVE('',#36887,#36888,#4270,.T.);
#45965=EDGE_CURVE('',#36888,#36889,#30574,.T.);
#45966=EDGE_CURVE('',#36889,#36890,#4271,.T.);
#45967=EDGE_CURVE('',#36890,#36891,#20126,.T.);
#45968=EDGE_CURVE('',#36891,#36892,#30575,.T.);
#45969=EDGE_CURVE('',#36892,#36893,#20127,.T.);
#45970=EDGE_CURVE('',#36893,#36894,#4272,.T.);
#45971=EDGE_CURVE('',#36894,#36895,#30576,.T.);
#45972=EDGE_CURVE('',#36895,#36896,#4273,.T.);
#45973=EDGE_CURVE('',#36896,#36897,#20128,.T.);
#45974=EDGE_CURVE('',#36897,#36898,#30577,.T.);
#45975=EDGE_CURVE('',#36898,#36899,#20129,.T.);
#45976=EDGE_CURVE('',#36899,#36900,#4274,.T.);
#45977=EDGE_CURVE('',#36900,#36901,#30578,.T.);
#45978=EDGE_CURVE('',#36901,#36902,#4275,.T.);
#45979=EDGE_CURVE('',#36902,#36903,#20130,.T.);
#45980=EDGE_CURVE('',#36903,#36904,#30579,.T.);
#45981=EDGE_CURVE('',#36904,#36905,#20131,.T.);
#45982=EDGE_CURVE('',#36905,#36906,#4276,.T.);
#45983=EDGE_CURVE('',#36906,#36907,#30580,.T.);
#45984=EDGE_CURVE('',#36907,#36908,#4277,.T.);
#45985=EDGE_CURVE('',#36908,#36909,#20132,.T.);
#45986=EDGE_CURVE('',#36909,#36910,#30581,.T.);
#45987=EDGE_CURVE('',#36910,#36911,#20133,.T.);
#45988=EDGE_CURVE('',#36911,#36912,#4278,.T.);
#45989=EDGE_CURVE('',#36912,#36913,#30582,.T.);
#45990=EDGE_CURVE('',#36913,#36914,#4279,.T.);
#45991=EDGE_CURVE('',#36914,#36915,#20134,.T.);
#45992=EDGE_CURVE('',#36915,#36916,#30583,.T.);
#45993=EDGE_CURVE('',#36916,#36917,#20135,.T.);
#45994=EDGE_CURVE('',#36917,#36918,#4280,.T.);
#45995=EDGE_CURVE('',#36918,#36919,#30584,.T.);
#45996=EDGE_CURVE('',#36919,#36920,#4281,.T.);
#45997=EDGE_CURVE('',#36920,#36921,#20136,.T.);
#45998=EDGE_CURVE('',#36921,#36922,#30585,.T.);
#45999=EDGE_CURVE('',#36922,#36923,#20137,.T.);
#46000=EDGE_CURVE('',#36923,#36924,#4282,.T.);
#46001=EDGE_CURVE('',#36924,#36925,#30586,.T.);
#46002=EDGE_CURVE('',#36925,#36926,#4283,.T.);
#46003=EDGE_CURVE('',#36926,#36927,#20138,.T.);
#46004=EDGE_CURVE('',#36927,#36928,#30587,.T.);
#46005=EDGE_CURVE('',#36928,#36929,#20139,.T.);
#46006=EDGE_CURVE('',#36929,#36930,#4284,.T.);
#46007=EDGE_CURVE('',#36930,#36931,#30588,.T.);
#46008=EDGE_CURVE('',#36931,#36932,#4285,.T.);
#46009=EDGE_CURVE('',#36932,#36933,#20140,.T.);
#46010=EDGE_CURVE('',#36933,#36934,#30589,.T.);
#46011=EDGE_CURVE('',#36934,#36935,#20141,.T.);
#46012=EDGE_CURVE('',#36935,#36936,#4286,.T.);
#46013=EDGE_CURVE('',#36936,#36937,#30590,.T.);
#46014=EDGE_CURVE('',#36937,#36938,#4287,.T.);
#46015=EDGE_CURVE('',#36938,#36939,#20142,.T.);
#46016=EDGE_CURVE('',#36939,#36940,#30591,.T.);
#46017=EDGE_CURVE('',#36940,#36941,#20143,.T.);
#46018=EDGE_CURVE('',#36941,#36942,#4288,.T.);
#46019=EDGE_CURVE('',#36942,#36943,#30592,.T.);
#46020=EDGE_CURVE('',#36943,#36944,#4289,.T.);
#46021=EDGE_CURVE('',#36944,#36945,#20144,.T.);
#46022=EDGE_CURVE('',#36945,#36946,#30593,.T.);
#46023=EDGE_CURVE('',#36946,#36947,#20145,.T.);
#46024=EDGE_CURVE('',#36947,#36948,#4290,.T.);
#46025=EDGE_CURVE('',#36948,#36949,#30594,.T.);
#46026=EDGE_CURVE('',#36949,#36950,#4291,.T.);
#46027=EDGE_CURVE('',#36950,#36951,#20146,.T.);
#46028=EDGE_CURVE('',#36951,#36952,#30595,.T.);
#46029=EDGE_CURVE('',#36952,#36953,#20147,.T.);
#46030=EDGE_CURVE('',#36953,#36954,#4292,.T.);
#46031=EDGE_CURVE('',#36954,#36955,#30596,.T.);
#46032=EDGE_CURVE('',#36955,#36956,#4293,.T.);
#46033=EDGE_CURVE('',#36956,#36957,#20148,.T.);
#46034=EDGE_CURVE('',#36957,#36958,#30597,.T.);
#46035=EDGE_CURVE('',#36958,#36959,#20149,.T.);
#46036=EDGE_CURVE('',#36959,#36960,#4294,.T.);
#46037=EDGE_CURVE('',#36960,#36961,#30598,.T.);
#46038=EDGE_CURVE('',#36961,#36962,#4295,.T.);
#46039=EDGE_CURVE('',#36962,#36963,#20150,.T.);
#46040=EDGE_CURVE('',#36963,#36964,#30599,.T.);
#46041=EDGE_CURVE('',#36964,#36965,#20151,.T.);
#46042=EDGE_CURVE('',#36965,#36966,#4296,.T.);
#46043=EDGE_CURVE('',#36966,#36967,#30600,.T.);
#46044=EDGE_CURVE('',#36967,#36968,#4297,.T.);
#46045=EDGE_CURVE('',#36968,#36969,#20152,.T.);
#46046=EDGE_CURVE('',#36969,#36970,#30601,.T.);
#46047=EDGE_CURVE('',#36970,#36971,#20153,.T.);
#46048=EDGE_CURVE('',#36971,#36972,#4298,.T.);
#46049=EDGE_CURVE('',#36972,#36973,#30602,.T.);
#46050=EDGE_CURVE('',#36973,#36974,#4299,.T.);
#46051=EDGE_CURVE('',#36974,#36975,#20154,.T.);
#46052=EDGE_CURVE('',#36975,#36976,#30603,.T.);
#46053=EDGE_CURVE('',#36976,#36977,#20155,.T.);
#46054=EDGE_CURVE('',#36977,#36978,#4300,.T.);
#46055=EDGE_CURVE('',#36978,#36979,#30604,.T.);
#46056=EDGE_CURVE('',#36979,#36980,#4301,.T.);
#46057=EDGE_CURVE('',#36980,#36981,#20156,.T.);
#46058=EDGE_CURVE('',#36981,#36982,#30605,.T.);
#46059=EDGE_CURVE('',#36982,#36983,#20157,.T.);
#46060=EDGE_CURVE('',#36983,#36984,#4302,.T.);
#46061=EDGE_CURVE('',#36984,#36985,#30606,.T.);
#46062=EDGE_CURVE('',#36985,#36986,#4303,.T.);
#46063=EDGE_CURVE('',#36986,#36987,#20158,.T.);
#46064=EDGE_CURVE('',#36987,#36988,#30607,.T.);
#46065=EDGE_CURVE('',#36988,#36989,#20159,.T.);
#46066=EDGE_CURVE('',#36989,#36990,#4304,.T.);
#46067=EDGE_CURVE('',#36990,#36991,#30608,.T.);
#46068=EDGE_CURVE('',#36991,#36992,#4305,.T.);
#46069=EDGE_CURVE('',#36992,#36993,#20160,.T.);
#46070=EDGE_CURVE('',#36993,#36994,#30609,.T.);
#46071=EDGE_CURVE('',#36994,#36995,#20161,.T.);
#46072=EDGE_CURVE('',#36995,#36996,#4306,.T.);
#46073=EDGE_CURVE('',#36996,#36997,#30610,.T.);
#46074=EDGE_CURVE('',#36997,#36998,#4307,.T.);
#46075=EDGE_CURVE('',#36998,#36999,#20162,.T.);
#46076=EDGE_CURVE('',#36999,#37000,#30611,.T.);
#46077=EDGE_CURVE('',#37000,#37001,#20163,.T.);
#46078=EDGE_CURVE('',#37001,#37002,#4308,.T.);
#46079=EDGE_CURVE('',#37002,#37003,#30612,.T.);
#46080=EDGE_CURVE('',#37003,#37004,#4309,.T.);
#46081=EDGE_CURVE('',#37004,#37005,#20164,.T.);
#46082=EDGE_CURVE('',#37005,#37006,#30613,.T.);
#46083=EDGE_CURVE('',#37006,#37007,#20165,.T.);
#46084=EDGE_CURVE('',#37007,#37008,#4310,.T.);
#46085=EDGE_CURVE('',#37008,#37009,#30614,.T.);
#46086=EDGE_CURVE('',#37009,#37010,#4311,.T.);
#46087=EDGE_CURVE('',#37010,#37011,#20166,.T.);
#46088=EDGE_CURVE('',#37011,#37012,#30615,.T.);
#46089=EDGE_CURVE('',#37012,#37013,#20167,.T.);
#46090=EDGE_CURVE('',#37013,#37014,#4312,.T.);
#46091=EDGE_CURVE('',#37014,#37015,#30616,.T.);
#46092=EDGE_CURVE('',#37015,#37016,#4313,.T.);
#46093=EDGE_CURVE('',#37016,#37017,#20168,.T.);
#46094=EDGE_CURVE('',#37017,#37018,#30617,.T.);
#46095=EDGE_CURVE('',#37018,#37019,#20169,.T.);
#46096=EDGE_CURVE('',#37019,#36823,#4314,.T.);
#46097=EDGE_CURVE('',#36824,#36835,#20170,.T.);
#46098=EDGE_CURVE('',#36827,#37020,#4315,.T.);
#46099=EDGE_CURVE('',#37020,#37021,#20171,.T.);
#46100=EDGE_CURVE('',#37021,#37022,#30618,.T.);
#46101=EDGE_CURVE('',#37022,#37023,#20172,.T.);
#46102=EDGE_CURVE('',#37023,#37024,#4316,.T.);
#46103=EDGE_CURVE('',#37024,#37025,#30619,.T.);
#46104=EDGE_CURVE('',#37025,#37026,#4317,.T.);
#46105=EDGE_CURVE('',#37026,#37027,#20173,.T.);
#46106=EDGE_CURVE('',#37027,#37028,#30620,.T.);
#46107=EDGE_CURVE('',#37028,#37029,#20174,.T.);
#46108=EDGE_CURVE('',#37029,#37030,#4318,.T.);
#46109=EDGE_CURVE('',#37030,#37031,#30621,.T.);
#46110=EDGE_CURVE('',#37031,#37032,#4319,.T.);
#46111=EDGE_CURVE('',#37032,#37033,#20175,.T.);
#46112=EDGE_CURVE('',#37033,#37034,#30622,.T.);
#46113=EDGE_CURVE('',#37034,#37035,#20176,.T.);
#46114=EDGE_CURVE('',#37035,#37036,#4320,.T.);
#46115=EDGE_CURVE('',#37036,#37037,#30623,.T.);
#46116=EDGE_CURVE('',#37037,#37038,#4321,.T.);
#46117=EDGE_CURVE('',#37038,#37039,#20177,.T.);
#46118=EDGE_CURVE('',#37039,#37040,#30624,.T.);
#46119=EDGE_CURVE('',#37040,#37041,#20178,.T.);
#46120=EDGE_CURVE('',#37041,#37042,#4322,.T.);
#46121=EDGE_CURVE('',#37042,#37043,#30625,.T.);
#46122=EDGE_CURVE('',#37043,#37044,#4323,.T.);
#46123=EDGE_CURVE('',#37044,#37045,#20179,.T.);
#46124=EDGE_CURVE('',#37045,#37046,#30626,.T.);
#46125=EDGE_CURVE('',#37046,#37047,#20180,.T.);
#46126=EDGE_CURVE('',#37047,#37048,#4324,.T.);
#46127=EDGE_CURVE('',#37048,#37049,#30627,.T.);
#46128=EDGE_CURVE('',#37049,#37050,#4325,.T.);
#46129=EDGE_CURVE('',#37050,#37051,#20181,.T.);
#46130=EDGE_CURVE('',#37051,#37052,#30628,.T.);
#46131=EDGE_CURVE('',#37052,#37053,#20182,.T.);
#46132=EDGE_CURVE('',#37053,#37054,#4326,.T.);
#46133=EDGE_CURVE('',#37054,#37055,#30629,.T.);
#46134=EDGE_CURVE('',#37055,#37056,#4327,.T.);
#46135=EDGE_CURVE('',#37056,#37057,#20183,.T.);
#46136=EDGE_CURVE('',#37057,#37058,#30630,.T.);
#46137=EDGE_CURVE('',#37058,#37059,#20184,.T.);
#46138=EDGE_CURVE('',#37059,#37060,#4328,.T.);
#46139=EDGE_CURVE('',#37060,#37061,#30631,.T.);
#46140=EDGE_CURVE('',#37061,#37062,#4329,.T.);
#46141=EDGE_CURVE('',#37062,#37063,#20185,.T.);
#46142=EDGE_CURVE('',#37063,#37064,#30632,.T.);
#46143=EDGE_CURVE('',#37064,#37065,#20186,.T.);
#46144=EDGE_CURVE('',#37065,#37066,#4330,.T.);
#46145=EDGE_CURVE('',#37066,#37067,#30633,.T.);
#46146=EDGE_CURVE('',#37067,#37068,#4331,.T.);
#46147=EDGE_CURVE('',#37068,#37069,#20187,.T.);
#46148=EDGE_CURVE('',#37069,#37070,#30634,.T.);
#46149=EDGE_CURVE('',#37070,#37071,#20188,.T.);
#46150=EDGE_CURVE('',#37071,#37072,#4332,.T.);
#46151=EDGE_CURVE('',#37072,#37073,#30635,.T.);
#46152=EDGE_CURVE('',#37073,#37074,#4333,.T.);
#46153=EDGE_CURVE('',#37074,#37075,#20189,.T.);
#46154=EDGE_CURVE('',#37075,#37076,#30636,.T.);
#46155=EDGE_CURVE('',#37076,#37077,#20190,.T.);
#46156=EDGE_CURVE('',#37077,#37078,#4334,.T.);
#46157=EDGE_CURVE('',#37078,#37079,#30637,.T.);
#46158=EDGE_CURVE('',#37079,#37080,#4335,.T.);
#46159=EDGE_CURVE('',#37080,#37081,#20191,.T.);
#46160=EDGE_CURVE('',#37081,#37082,#30638,.T.);
#46161=EDGE_CURVE('',#37082,#37083,#20192,.T.);
#46162=EDGE_CURVE('',#37083,#37084,#4336,.T.);
#46163=EDGE_CURVE('',#37084,#37085,#30639,.T.);
#46164=EDGE_CURVE('',#37085,#37086,#4337,.T.);
#46165=EDGE_CURVE('',#37086,#37087,#20193,.T.);
#46166=EDGE_CURVE('',#37087,#37088,#30640,.T.);
#46167=EDGE_CURVE('',#37088,#37089,#20194,.T.);
#46168=EDGE_CURVE('',#37089,#37090,#4338,.T.);
#46169=EDGE_CURVE('',#37090,#37091,#30641,.T.);
#46170=EDGE_CURVE('',#37091,#37092,#4339,.T.);
#46171=EDGE_CURVE('',#37092,#37093,#20195,.T.);
#46172=EDGE_CURVE('',#37093,#37094,#30642,.T.);
#46173=EDGE_CURVE('',#37094,#37095,#20196,.T.);
#46174=EDGE_CURVE('',#37095,#37096,#4340,.T.);
#46175=EDGE_CURVE('',#37096,#37097,#30643,.T.);
#46176=EDGE_CURVE('',#37097,#37098,#4341,.T.);
#46177=EDGE_CURVE('',#37098,#37099,#20197,.T.);
#46178=EDGE_CURVE('',#37099,#37100,#30644,.T.);
#46179=EDGE_CURVE('',#37100,#37101,#20198,.T.);
#46180=EDGE_CURVE('',#37101,#37102,#4342,.T.);
#46181=EDGE_CURVE('',#37102,#37103,#30645,.T.);
#46182=EDGE_CURVE('',#37103,#37104,#4343,.T.);
#46183=EDGE_CURVE('',#37104,#37105,#20199,.T.);
#46184=EDGE_CURVE('',#37105,#37106,#30646,.T.);
#46185=EDGE_CURVE('',#37106,#37107,#20200,.T.);
#46186=EDGE_CURVE('',#37107,#36815,#4344,.T.);
#46187=EDGE_CURVE('',#36816,#37108,#4345,.T.);
#46188=EDGE_CURVE('',#37108,#37109,#20201,.T.);
#46189=EDGE_CURVE('',#37109,#37110,#30647,.T.);
#46190=EDGE_CURVE('',#37110,#37111,#20202,.T.);
#46191=EDGE_CURVE('',#37111,#37112,#4346,.T.);
#46192=EDGE_CURVE('',#37112,#37113,#30648,.T.);
#46193=EDGE_CURVE('',#37113,#37114,#4347,.T.);
#46194=EDGE_CURVE('',#37114,#37115,#20203,.T.);
#46195=EDGE_CURVE('',#37115,#37116,#30649,.T.);
#46196=EDGE_CURVE('',#37116,#37117,#20204,.T.);
#46197=EDGE_CURVE('',#37117,#37118,#4348,.T.);
#46198=EDGE_CURVE('',#37118,#37119,#30650,.T.);
#46199=EDGE_CURVE('',#37119,#37120,#4349,.T.);
#46200=EDGE_CURVE('',#37120,#37121,#20205,.T.);
#46201=EDGE_CURVE('',#37121,#37122,#30651,.T.);
#46202=EDGE_CURVE('',#37122,#37123,#20206,.T.);
#46203=EDGE_CURVE('',#37123,#37124,#4350,.T.);
#46204=EDGE_CURVE('',#37124,#37125,#30652,.T.);
#46205=EDGE_CURVE('',#37125,#37126,#4351,.T.);
#46206=EDGE_CURVE('',#37126,#37127,#20207,.T.);
#46207=EDGE_CURVE('',#37127,#37128,#30653,.T.);
#46208=EDGE_CURVE('',#37128,#37129,#20208,.T.);
#46209=EDGE_CURVE('',#37129,#37130,#4352,.T.);
#46210=EDGE_CURVE('',#37130,#37131,#30654,.T.);
#46211=EDGE_CURVE('',#37131,#37132,#4353,.T.);
#46212=EDGE_CURVE('',#37132,#37133,#20209,.T.);
#46213=EDGE_CURVE('',#37133,#37134,#30655,.T.);
#46214=EDGE_CURVE('',#37134,#37135,#20210,.T.);
#46215=EDGE_CURVE('',#37135,#37136,#4354,.T.);
#46216=EDGE_CURVE('',#37136,#37137,#30656,.T.);
#46217=EDGE_CURVE('',#37137,#37138,#4355,.T.);
#46218=EDGE_CURVE('',#37138,#37139,#20211,.T.);
#46219=EDGE_CURVE('',#37139,#37140,#30657,.T.);
#46220=EDGE_CURVE('',#37140,#37141,#20212,.T.);
#46221=EDGE_CURVE('',#37141,#37142,#4356,.T.);
#46222=EDGE_CURVE('',#37142,#37143,#30658,.T.);
#46223=EDGE_CURVE('',#37143,#37144,#4357,.T.);
#46224=EDGE_CURVE('',#37144,#37145,#20213,.T.);
#46225=EDGE_CURVE('',#37145,#37146,#30659,.T.);
#46226=EDGE_CURVE('',#37146,#37147,#20214,.T.);
#46227=EDGE_CURVE('',#37147,#37148,#4358,.T.);
#46228=EDGE_CURVE('',#37148,#37149,#30660,.T.);
#46229=EDGE_CURVE('',#37149,#37150,#4359,.T.);
#46230=EDGE_CURVE('',#37150,#37151,#20215,.T.);
#46231=EDGE_CURVE('',#37151,#37152,#30661,.T.);
#46232=EDGE_CURVE('',#37152,#37153,#20216,.T.);
#46233=EDGE_CURVE('',#37153,#37154,#4360,.T.);
#46234=EDGE_CURVE('',#37154,#37155,#30662,.T.);
#46235=EDGE_CURVE('',#37155,#37156,#4361,.T.);
#46236=EDGE_CURVE('',#37156,#37157,#20217,.T.);
#46237=EDGE_CURVE('',#37157,#37158,#30663,.T.);
#46238=EDGE_CURVE('',#37158,#37159,#20218,.T.);
#46239=EDGE_CURVE('',#37159,#37160,#4362,.T.);
#46240=EDGE_CURVE('',#37160,#37161,#30664,.T.);
#46241=EDGE_CURVE('',#37161,#37162,#4363,.T.);
#46242=EDGE_CURVE('',#37162,#37163,#20219,.T.);
#46243=EDGE_CURVE('',#37163,#37164,#30665,.T.);
#46244=EDGE_CURVE('',#37164,#37165,#20220,.T.);
#46245=EDGE_CURVE('',#37165,#37166,#4364,.T.);
#46246=EDGE_CURVE('',#37166,#37167,#30666,.T.);
#46247=EDGE_CURVE('',#37167,#37168,#4365,.T.);
#46248=EDGE_CURVE('',#37168,#37169,#20221,.T.);
#46249=EDGE_CURVE('',#37169,#37170,#30667,.T.);
#46250=EDGE_CURVE('',#37170,#37171,#20222,.T.);
#46251=EDGE_CURVE('',#37171,#37172,#4366,.T.);
#46252=EDGE_CURVE('',#37172,#37173,#30668,.T.);
#46253=EDGE_CURVE('',#37173,#37174,#4367,.T.);
#46254=EDGE_CURVE('',#37174,#37175,#20223,.T.);
#46255=EDGE_CURVE('',#37175,#37176,#30669,.T.);
#46256=EDGE_CURVE('',#37176,#37177,#20224,.T.);
#46257=EDGE_CURVE('',#37177,#37178,#4368,.T.);
#46258=EDGE_CURVE('',#37178,#37179,#30670,.T.);
#46259=EDGE_CURVE('',#37179,#37180,#4369,.T.);
#46260=EDGE_CURVE('',#37180,#37181,#20225,.T.);
#46261=EDGE_CURVE('',#37181,#37182,#30671,.T.);
#46262=EDGE_CURVE('',#37182,#37183,#20226,.T.);
#46263=EDGE_CURVE('',#37183,#37184,#4370,.T.);
#46264=EDGE_CURVE('',#37184,#37185,#30672,.T.);
#46265=EDGE_CURVE('',#37185,#37186,#4371,.T.);
#46266=EDGE_CURVE('',#37186,#37187,#20227,.T.);
#46267=EDGE_CURVE('',#37187,#37188,#30673,.T.);
#46268=EDGE_CURVE('',#37188,#37189,#20228,.T.);
#46269=EDGE_CURVE('',#37189,#37190,#4372,.T.);
#46270=EDGE_CURVE('',#37190,#37191,#30674,.T.);
#46271=EDGE_CURVE('',#37191,#37192,#4373,.T.);
#46272=EDGE_CURVE('',#37192,#37193,#20229,.T.);
#46273=EDGE_CURVE('',#37193,#37194,#30675,.T.);
#46274=EDGE_CURVE('',#37194,#37195,#20230,.T.);
#46275=EDGE_CURVE('',#37195,#36840,#4374,.T.);
#46276=EDGE_CURVE('',#36821,#37196,#4375,.T.);
#46277=EDGE_CURVE('',#37196,#37197,#20231,.T.);
#46278=EDGE_CURVE('',#37197,#37198,#30676,.T.);
#46279=EDGE_CURVE('',#37198,#37199,#20232,.T.);
#46280=EDGE_CURVE('',#37199,#37200,#4376,.T.);
#46281=EDGE_CURVE('',#37200,#37201,#30677,.T.);
#46282=EDGE_CURVE('',#37201,#37202,#4377,.T.);
#46283=EDGE_CURVE('',#37202,#37203,#20233,.T.);
#46284=EDGE_CURVE('',#37203,#37204,#30678,.T.);
#46285=EDGE_CURVE('',#37204,#37205,#20234,.T.);
#46286=EDGE_CURVE('',#37205,#37206,#4378,.T.);
#46287=EDGE_CURVE('',#37206,#37207,#30679,.T.);
#46288=EDGE_CURVE('',#37207,#37208,#4379,.T.);
#46289=EDGE_CURVE('',#37208,#37209,#20235,.T.);
#46290=EDGE_CURVE('',#37209,#37210,#30680,.T.);
#46291=EDGE_CURVE('',#37210,#37211,#20236,.T.);
#46292=EDGE_CURVE('',#37211,#37212,#4380,.T.);
#46293=EDGE_CURVE('',#37212,#37213,#30681,.T.);
#46294=EDGE_CURVE('',#37213,#37214,#4381,.T.);
#46295=EDGE_CURVE('',#37214,#37215,#20237,.T.);
#46296=EDGE_CURVE('',#37215,#37216,#30682,.T.);
#46297=EDGE_CURVE('',#37216,#37217,#20238,.T.);
#46298=EDGE_CURVE('',#37217,#37218,#4382,.T.);
#46299=EDGE_CURVE('',#37218,#37219,#30683,.T.);
#46300=EDGE_CURVE('',#37219,#37220,#4383,.T.);
#46301=EDGE_CURVE('',#37220,#37221,#20239,.T.);
#46302=EDGE_CURVE('',#37221,#37222,#30684,.T.);
#46303=EDGE_CURVE('',#37222,#37223,#20240,.T.);
#46304=EDGE_CURVE('',#37223,#37224,#4384,.T.);
#46305=EDGE_CURVE('',#37224,#37225,#30685,.T.);
#46306=EDGE_CURVE('',#37225,#37226,#4385,.T.);
#46307=EDGE_CURVE('',#37226,#37227,#20241,.T.);
#46308=EDGE_CURVE('',#37227,#37228,#30686,.T.);
#46309=EDGE_CURVE('',#37228,#37229,#20242,.T.);
#46310=EDGE_CURVE('',#37229,#37230,#4386,.T.);
#46311=EDGE_CURVE('',#37230,#37231,#30687,.T.);
#46312=EDGE_CURVE('',#37231,#37232,#4387,.T.);
#46313=EDGE_CURVE('',#37232,#37233,#20243,.T.);
#46314=EDGE_CURVE('',#37233,#37234,#30688,.T.);
#46315=EDGE_CURVE('',#37234,#37235,#20244,.T.);
#46316=EDGE_CURVE('',#37235,#37236,#4388,.T.);
#46317=EDGE_CURVE('',#37236,#37237,#30689,.T.);
#46318=EDGE_CURVE('',#37237,#37238,#4389,.T.);
#46319=EDGE_CURVE('',#37238,#37239,#20245,.T.);
#46320=EDGE_CURVE('',#37239,#37240,#30690,.T.);
#46321=EDGE_CURVE('',#37240,#37241,#20246,.T.);
#46322=EDGE_CURVE('',#37241,#37242,#4390,.T.);
#46323=EDGE_CURVE('',#37242,#37243,#30691,.T.);
#46324=EDGE_CURVE('',#37243,#37244,#4391,.T.);
#46325=EDGE_CURVE('',#37244,#37245,#20247,.T.);
#46326=EDGE_CURVE('',#37245,#37246,#30692,.T.);
#46327=EDGE_CURVE('',#37246,#37247,#20248,.T.);
#46328=EDGE_CURVE('',#37247,#37248,#4392,.T.);
#46329=EDGE_CURVE('',#37248,#37249,#30693,.T.);
#46330=EDGE_CURVE('',#37249,#37250,#4393,.T.);
#46331=EDGE_CURVE('',#37250,#37251,#20249,.T.);
#46332=EDGE_CURVE('',#37251,#37252,#30694,.T.);
#46333=EDGE_CURVE('',#37252,#37253,#20250,.T.);
#46334=EDGE_CURVE('',#37253,#37254,#4394,.T.);
#46335=EDGE_CURVE('',#37254,#37255,#30695,.T.);
#46336=EDGE_CURVE('',#37255,#37256,#4395,.T.);
#46337=EDGE_CURVE('',#37256,#37257,#20251,.T.);
#46338=EDGE_CURVE('',#37257,#37258,#30696,.T.);
#46339=EDGE_CURVE('',#37258,#37259,#20252,.T.);
#46340=EDGE_CURVE('',#37259,#37260,#4396,.T.);
#46341=EDGE_CURVE('',#37260,#37261,#30697,.T.);
#46342=EDGE_CURVE('',#37261,#37262,#4397,.T.);
#46343=EDGE_CURVE('',#37262,#37263,#20253,.T.);
#46344=EDGE_CURVE('',#37263,#37264,#30698,.T.);
#46345=EDGE_CURVE('',#37264,#37265,#20254,.T.);
#46346=EDGE_CURVE('',#37265,#37266,#4398,.T.);
#46347=EDGE_CURVE('',#37266,#37267,#30699,.T.);
#46348=EDGE_CURVE('',#37267,#37268,#4399,.T.);
#46349=EDGE_CURVE('',#37268,#37269,#20255,.T.);
#46350=EDGE_CURVE('',#37269,#37270,#30700,.T.);
#46351=EDGE_CURVE('',#37270,#37271,#20256,.T.);
#46352=EDGE_CURVE('',#37271,#37272,#4400,.T.);
#46353=EDGE_CURVE('',#37272,#37273,#30701,.T.);
#46354=EDGE_CURVE('',#37273,#37274,#4401,.T.);
#46355=EDGE_CURVE('',#37274,#37275,#20257,.T.);
#46356=EDGE_CURVE('',#37275,#37276,#30702,.T.);
#46357=EDGE_CURVE('',#37276,#37277,#20258,.T.);
#46358=EDGE_CURVE('',#37277,#37278,#4402,.T.);
#46359=EDGE_CURVE('',#37278,#37279,#30703,.T.);
#46360=EDGE_CURVE('',#37279,#37280,#4403,.T.);
#46361=EDGE_CURVE('',#37280,#37281,#20259,.T.);
#46362=EDGE_CURVE('',#37281,#37282,#30704,.T.);
#46363=EDGE_CURVE('',#37282,#37283,#20260,.T.);
#46364=EDGE_CURVE('',#37283,#37284,#4404,.T.);
#46365=EDGE_CURVE('',#37284,#37285,#30705,.T.);
#46366=EDGE_CURVE('',#37285,#37286,#4405,.T.);
#46367=EDGE_CURVE('',#37286,#37287,#20261,.T.);
#46368=EDGE_CURVE('',#37287,#37288,#30706,.T.);
#46369=EDGE_CURVE('',#37288,#37289,#20262,.T.);
#46370=EDGE_CURVE('',#37289,#37290,#4406,.T.);
#46371=EDGE_CURVE('',#37290,#37291,#30707,.T.);
#46372=EDGE_CURVE('',#37291,#37292,#4407,.T.);
#46373=EDGE_CURVE('',#37292,#37293,#20263,.T.);
#46374=EDGE_CURVE('',#37293,#37294,#30708,.T.);
#46375=EDGE_CURVE('',#37294,#37295,#20264,.T.);
#46376=EDGE_CURVE('',#37295,#37296,#4408,.T.);
#46377=EDGE_CURVE('',#37296,#37297,#30709,.T.);
#46378=EDGE_CURVE('',#37297,#37298,#4409,.T.);
#46379=EDGE_CURVE('',#37298,#37299,#20265,.T.);
#46380=EDGE_CURVE('',#37299,#37300,#30710,.T.);
#46381=EDGE_CURVE('',#37300,#37301,#20266,.T.);
#46382=EDGE_CURVE('',#37301,#37302,#4410,.T.);
#46383=EDGE_CURVE('',#37302,#37303,#30711,.T.);
#46384=EDGE_CURVE('',#37303,#37304,#4411,.T.);
#46385=EDGE_CURVE('',#37304,#37305,#20267,.T.);
#46386=EDGE_CURVE('',#37305,#37306,#30712,.T.);
#46387=EDGE_CURVE('',#37306,#37307,#20268,.T.);
#46388=EDGE_CURVE('',#37307,#37308,#4412,.T.);
#46389=EDGE_CURVE('',#37308,#37309,#30713,.T.);
#46390=EDGE_CURVE('',#37309,#37310,#4413,.T.);
#46391=EDGE_CURVE('',#37310,#37311,#20269,.T.);
#46392=EDGE_CURVE('',#37311,#37312,#30714,.T.);
#46393=EDGE_CURVE('',#37312,#37313,#20270,.T.);
#46394=EDGE_CURVE('',#37313,#37314,#4414,.T.);
#46395=EDGE_CURVE('',#37314,#37315,#30715,.T.);
#46396=EDGE_CURVE('',#37315,#37316,#4415,.T.);
#46397=EDGE_CURVE('',#37316,#37317,#20271,.T.);
#46398=EDGE_CURVE('',#37317,#37318,#30716,.T.);
#46399=EDGE_CURVE('',#37318,#37319,#20272,.T.);
#46400=EDGE_CURVE('',#37319,#37320,#4416,.T.);
#46401=EDGE_CURVE('',#37320,#37321,#30717,.T.);
#46402=EDGE_CURVE('',#37321,#37322,#4417,.T.);
#46403=EDGE_CURVE('',#37322,#37323,#20273,.T.);
#46404=EDGE_CURVE('',#37323,#37324,#30718,.T.);
#46405=EDGE_CURVE('',#37324,#37325,#20274,.T.);
#46406=EDGE_CURVE('',#37325,#37326,#4418,.T.);
#46407=EDGE_CURVE('',#37326,#37327,#30719,.T.);
#46408=EDGE_CURVE('',#37327,#37328,#4419,.T.);
#46409=EDGE_CURVE('',#37328,#37329,#20275,.T.);
#46410=EDGE_CURVE('',#37329,#37330,#30720,.T.);
#46411=EDGE_CURVE('',#37330,#37331,#20276,.T.);
#46412=EDGE_CURVE('',#37331,#37332,#4420,.T.);
#46413=EDGE_CURVE('',#37332,#37333,#30721,.T.);
#46414=EDGE_CURVE('',#37333,#37334,#4421,.T.);
#46415=EDGE_CURVE('',#37334,#37335,#20277,.T.);
#46416=EDGE_CURVE('',#37335,#37336,#30722,.T.);
#46417=EDGE_CURVE('',#37336,#37337,#20278,.T.);
#46418=EDGE_CURVE('',#37337,#37338,#4422,.T.);
#46419=EDGE_CURVE('',#37338,#37339,#30723,.T.);
#46420=EDGE_CURVE('',#37339,#37340,#4423,.T.);
#46421=EDGE_CURVE('',#37340,#37341,#20279,.T.);
#46422=EDGE_CURVE('',#37341,#37342,#30724,.T.);
#46423=EDGE_CURVE('',#37342,#37343,#20280,.T.);
#46424=EDGE_CURVE('',#37343,#37344,#4424,.T.);
#46425=EDGE_CURVE('',#37344,#37345,#30725,.T.);
#46426=EDGE_CURVE('',#37345,#37346,#4425,.T.);
#46427=EDGE_CURVE('',#37346,#37347,#20281,.T.);
#46428=EDGE_CURVE('',#37347,#37348,#30726,.T.);
#46429=EDGE_CURVE('',#37348,#37349,#20282,.T.);
#46430=EDGE_CURVE('',#37349,#37350,#4426,.T.);
#46431=EDGE_CURVE('',#37350,#37351,#30727,.T.);
#46432=EDGE_CURVE('',#37351,#37352,#4427,.T.);
#46433=EDGE_CURVE('',#37352,#37353,#20283,.T.);
#46434=EDGE_CURVE('',#37353,#37354,#30728,.T.);
#46435=EDGE_CURVE('',#37354,#37355,#20284,.T.);
#46436=EDGE_CURVE('',#37355,#37356,#4428,.T.);
#46437=EDGE_CURVE('',#37356,#37357,#30729,.T.);
#46438=EDGE_CURVE('',#37357,#37358,#4429,.T.);
#46439=EDGE_CURVE('',#37358,#37359,#20285,.T.);
#46440=EDGE_CURVE('',#37359,#37360,#30730,.T.);
#46441=EDGE_CURVE('',#37360,#37361,#20286,.T.);
#46442=EDGE_CURVE('',#37361,#37362,#4430,.T.);
#46443=EDGE_CURVE('',#37362,#37363,#30731,.T.);
#46444=EDGE_CURVE('',#37363,#37364,#4431,.T.);
#46445=EDGE_CURVE('',#37364,#37365,#20287,.T.);
#46446=EDGE_CURVE('',#37365,#37366,#30732,.T.);
#46447=EDGE_CURVE('',#37366,#37367,#20288,.T.);
#46448=EDGE_CURVE('',#37367,#37368,#4432,.T.);
#46449=EDGE_CURVE('',#37368,#37369,#30733,.T.);
#46450=EDGE_CURVE('',#37369,#37370,#4433,.T.);
#46451=EDGE_CURVE('',#37370,#37371,#20289,.T.);
#46452=EDGE_CURVE('',#37371,#37372,#30734,.T.);
#46453=EDGE_CURVE('',#37372,#37373,#20290,.T.);
#46454=EDGE_CURVE('',#37373,#37374,#4434,.T.);
#46455=EDGE_CURVE('',#37374,#37375,#30735,.T.);
#46456=EDGE_CURVE('',#37375,#36831,#20291,.T.);
#46457=EDGE_CURVE('',#37375,#37376,#30736,.T.);
#46458=EDGE_CURVE('',#37376,#37377,#4435,.T.);
#46459=EDGE_CURVE('',#37377,#37378,#20292,.T.);
#46460=EDGE_CURVE('',#37378,#37379,#30737,.T.);
#46461=EDGE_CURVE('',#37379,#37380,#20293,.T.);
#46462=EDGE_CURVE('',#37380,#37381,#4436,.T.);
#46463=EDGE_CURVE('',#37381,#37382,#30738,.T.);
#46464=EDGE_CURVE('',#37382,#37383,#4437,.T.);
#46465=EDGE_CURVE('',#37383,#37384,#20294,.T.);
#46466=EDGE_CURVE('',#37384,#37385,#30739,.T.);
#46467=EDGE_CURVE('',#37385,#37386,#20295,.T.);
#46468=EDGE_CURVE('',#37386,#37387,#4438,.T.);
#46469=EDGE_CURVE('',#37387,#37388,#30740,.T.);
#46470=EDGE_CURVE('',#37388,#37389,#4439,.T.);
#46471=EDGE_CURVE('',#37389,#37390,#20296,.T.);
#46472=EDGE_CURVE('',#37390,#37391,#30741,.T.);
#46473=EDGE_CURVE('',#37391,#37392,#20297,.T.);
#46474=EDGE_CURVE('',#37392,#37393,#4440,.T.);
#46475=EDGE_CURVE('',#37393,#37394,#30742,.T.);
#46476=EDGE_CURVE('',#37394,#37395,#4441,.T.);
#46477=EDGE_CURVE('',#37395,#37396,#20298,.T.);
#46478=EDGE_CURVE('',#37396,#37397,#30743,.T.);
#46479=EDGE_CURVE('',#37397,#37398,#20299,.T.);
#46480=EDGE_CURVE('',#37398,#37399,#4442,.T.);
#46481=EDGE_CURVE('',#37399,#37400,#30744,.T.);
#46482=EDGE_CURVE('',#37400,#37401,#4443,.T.);
#46483=EDGE_CURVE('',#37401,#37402,#20300,.T.);
#46484=EDGE_CURVE('',#37402,#37403,#30745,.T.);
#46485=EDGE_CURVE('',#37403,#37404,#20301,.T.);
#46486=EDGE_CURVE('',#37404,#37405,#4444,.T.);
#46487=EDGE_CURVE('',#37405,#37406,#30746,.T.);
#46488=EDGE_CURVE('',#37406,#37407,#4445,.T.);
#46489=EDGE_CURVE('',#37407,#37408,#20302,.T.);
#46490=EDGE_CURVE('',#37408,#37409,#30747,.T.);
#46491=EDGE_CURVE('',#37409,#37410,#20303,.T.);
#46492=EDGE_CURVE('',#37410,#37411,#4446,.T.);
#46493=EDGE_CURVE('',#37411,#37412,#30748,.T.);
#46494=EDGE_CURVE('',#37412,#37413,#4447,.T.);
#46495=EDGE_CURVE('',#37413,#37414,#20304,.T.);
#46496=EDGE_CURVE('',#37414,#37415,#30749,.T.);
#46497=EDGE_CURVE('',#37415,#37416,#20305,.T.);
#46498=EDGE_CURVE('',#37416,#37417,#4448,.T.);
#46499=EDGE_CURVE('',#37417,#37418,#30750,.T.);
#46500=EDGE_CURVE('',#37418,#37419,#4449,.T.);
#46501=EDGE_CURVE('',#37419,#37420,#20306,.T.);
#46502=EDGE_CURVE('',#37420,#37421,#30751,.T.);
#46503=EDGE_CURVE('',#37421,#37422,#20307,.T.);
#46504=EDGE_CURVE('',#37422,#37423,#4450,.T.);
#46505=EDGE_CURVE('',#37423,#37424,#30752,.T.);
#46506=EDGE_CURVE('',#37424,#37425,#4451,.T.);
#46507=EDGE_CURVE('',#37425,#37426,#20308,.T.);
#46508=EDGE_CURVE('',#37426,#37427,#30753,.T.);
#46509=EDGE_CURVE('',#37427,#37428,#20309,.T.);
#46510=EDGE_CURVE('',#37428,#37429,#4452,.T.);
#46511=EDGE_CURVE('',#37429,#37430,#30754,.T.);
#46512=EDGE_CURVE('',#37430,#37431,#4453,.T.);
#46513=EDGE_CURVE('',#37431,#37432,#20310,.T.);
#46514=EDGE_CURVE('',#37432,#37433,#30755,.T.);
#46515=EDGE_CURVE('',#37433,#37434,#20311,.T.);
#46516=EDGE_CURVE('',#37434,#37435,#4454,.T.);
#46517=EDGE_CURVE('',#37435,#37436,#30756,.T.);
#46518=EDGE_CURVE('',#37436,#37437,#4455,.T.);
#46519=EDGE_CURVE('',#37437,#37438,#20312,.T.);
#46520=EDGE_CURVE('',#37438,#37439,#30757,.T.);
#46521=EDGE_CURVE('',#37439,#37440,#20313,.T.);
#46522=EDGE_CURVE('',#37440,#37441,#4456,.T.);
#46523=EDGE_CURVE('',#37441,#37442,#30758,.T.);
#46524=EDGE_CURVE('',#37442,#37443,#4457,.T.);
#46525=EDGE_CURVE('',#37443,#37444,#20314,.T.);
#46526=EDGE_CURVE('',#37444,#37445,#30759,.T.);
#46527=EDGE_CURVE('',#37445,#37446,#20315,.T.);
#46528=EDGE_CURVE('',#37446,#37447,#4458,.T.);
#46529=EDGE_CURVE('',#37447,#37448,#30760,.T.);
#46530=EDGE_CURVE('',#37448,#37449,#4459,.T.);
#46531=EDGE_CURVE('',#37449,#37450,#20316,.T.);
#46532=EDGE_CURVE('',#37450,#37451,#30761,.T.);
#46533=EDGE_CURVE('',#37451,#37452,#20317,.T.);
#46534=EDGE_CURVE('',#37452,#37453,#4460,.T.);
#46535=EDGE_CURVE('',#37453,#37454,#30762,.T.);
#46536=EDGE_CURVE('',#37454,#37455,#4461,.T.);
#46537=EDGE_CURVE('',#37455,#37456,#20318,.T.);
#46538=EDGE_CURVE('',#37456,#37457,#30763,.T.);
#46539=EDGE_CURVE('',#37457,#37458,#20319,.T.);
#46540=EDGE_CURVE('',#37458,#37459,#4462,.T.);
#46541=EDGE_CURVE('',#37459,#37460,#30764,.T.);
#46542=EDGE_CURVE('',#37460,#37461,#4463,.T.);
#46543=EDGE_CURVE('',#37461,#37462,#20320,.T.);
#46544=EDGE_CURVE('',#37462,#37463,#30765,.T.);
#46545=EDGE_CURVE('',#37463,#37464,#20321,.T.);
#46546=EDGE_CURVE('',#37464,#36814,#4464,.T.);
#46547=EDGE_CURVE('',#36813,#37465,#4465,.T.);
#46548=EDGE_CURVE('',#37465,#37466,#20322,.T.);
#46549=EDGE_CURVE('',#37466,#37467,#30766,.T.);
#46550=EDGE_CURVE('',#37467,#37468,#20323,.T.);
#46551=EDGE_CURVE('',#37468,#37469,#4466,.T.);
#46552=EDGE_CURVE('',#37469,#37470,#30767,.T.);
#46553=EDGE_CURVE('',#37470,#37471,#4467,.T.);
#46554=EDGE_CURVE('',#37471,#37472,#20324,.T.);
#46555=EDGE_CURVE('',#37472,#37473,#30768,.T.);
#46556=EDGE_CURVE('',#37473,#37474,#20325,.T.);
#46557=EDGE_CURVE('',#37474,#37475,#4468,.T.);
#46558=EDGE_CURVE('',#37475,#37476,#30769,.T.);
#46559=EDGE_CURVE('',#37476,#37477,#4469,.T.);
#46560=EDGE_CURVE('',#37477,#37478,#20326,.T.);
#46561=EDGE_CURVE('',#37478,#37479,#30770,.T.);
#46562=EDGE_CURVE('',#37479,#37480,#20327,.T.);
#46563=EDGE_CURVE('',#37480,#37481,#4470,.T.);
#46564=EDGE_CURVE('',#37481,#37482,#30771,.T.);
#46565=EDGE_CURVE('',#37482,#37483,#4471,.T.);
#46566=EDGE_CURVE('',#37483,#37484,#20328,.T.);
#46567=EDGE_CURVE('',#37484,#37485,#30772,.T.);
#46568=EDGE_CURVE('',#37485,#37486,#20329,.T.);
#46569=EDGE_CURVE('',#37486,#37487,#4472,.T.);
#46570=EDGE_CURVE('',#37487,#37488,#30773,.T.);
#46571=EDGE_CURVE('',#37488,#37489,#4473,.T.);
#46572=EDGE_CURVE('',#37489,#37490,#20330,.T.);
#46573=EDGE_CURVE('',#37490,#37491,#30774,.T.);
#46574=EDGE_CURVE('',#37491,#37492,#20331,.T.);
#46575=EDGE_CURVE('',#37492,#37493,#4474,.T.);
#46576=EDGE_CURVE('',#37493,#37494,#30775,.T.);
#46577=EDGE_CURVE('',#37494,#37495,#4475,.T.);
#46578=EDGE_CURVE('',#37495,#37496,#20332,.T.);
#46579=EDGE_CURVE('',#37496,#37497,#30776,.T.);
#46580=EDGE_CURVE('',#37497,#37498,#20333,.T.);
#46581=EDGE_CURVE('',#37498,#37499,#4476,.T.);
#46582=EDGE_CURVE('',#37499,#37500,#30777,.T.);
#46583=EDGE_CURVE('',#37500,#37501,#4477,.T.);
#46584=EDGE_CURVE('',#37501,#37502,#20334,.T.);
#46585=EDGE_CURVE('',#37502,#37503,#30778,.T.);
#46586=EDGE_CURVE('',#37503,#37504,#20335,.T.);
#46587=EDGE_CURVE('',#37504,#37505,#4478,.T.);
#46588=EDGE_CURVE('',#37505,#37506,#30779,.T.);
#46589=EDGE_CURVE('',#37506,#37507,#4479,.T.);
#46590=EDGE_CURVE('',#37507,#37508,#20336,.T.);
#46591=EDGE_CURVE('',#37508,#37509,#30780,.T.);
#46592=EDGE_CURVE('',#37509,#37510,#20337,.T.);
#46593=EDGE_CURVE('',#37510,#37511,#4480,.T.);
#46594=EDGE_CURVE('',#37511,#37512,#30781,.T.);
#46595=EDGE_CURVE('',#37512,#37513,#4481,.T.);
#46596=EDGE_CURVE('',#37513,#37514,#20338,.T.);
#46597=EDGE_CURVE('',#37514,#37515,#30782,.T.);
#46598=EDGE_CURVE('',#37515,#37516,#20339,.T.);
#46599=EDGE_CURVE('',#37516,#37517,#4482,.T.);
#46600=EDGE_CURVE('',#37517,#37518,#30783,.T.);
#46601=EDGE_CURVE('',#37518,#37519,#4483,.T.);
#46602=EDGE_CURVE('',#37519,#37520,#20340,.T.);
#46603=EDGE_CURVE('',#37520,#37521,#30784,.T.);
#46604=EDGE_CURVE('',#37521,#37522,#20341,.T.);
#46605=EDGE_CURVE('',#37522,#37523,#4484,.T.);
#46606=EDGE_CURVE('',#37523,#37524,#30785,.T.);
#46607=EDGE_CURVE('',#37524,#37525,#4485,.T.);
#46608=EDGE_CURVE('',#37525,#37526,#20342,.T.);
#46609=EDGE_CURVE('',#37526,#37527,#30786,.T.);
#46610=EDGE_CURVE('',#37527,#37528,#20343,.T.);
#46611=EDGE_CURVE('',#37528,#37529,#4486,.T.);
#46612=EDGE_CURVE('',#37529,#37530,#30787,.T.);
#46613=EDGE_CURVE('',#37530,#37531,#4487,.T.);
#46614=EDGE_CURVE('',#37531,#37532,#20344,.T.);
#46615=EDGE_CURVE('',#37532,#37533,#30788,.T.);
#46616=EDGE_CURVE('',#37533,#37534,#20345,.T.);
#46617=EDGE_CURVE('',#37534,#37535,#4488,.T.);
#46618=EDGE_CURVE('',#37535,#37536,#30789,.T.);
#46619=EDGE_CURVE('',#37536,#37537,#4489,.T.);
#46620=EDGE_CURVE('',#37537,#37538,#20346,.T.);
#46621=EDGE_CURVE('',#37538,#37539,#30790,.T.);
#46622=EDGE_CURVE('',#37539,#37540,#20347,.T.);
#46623=EDGE_CURVE('',#37540,#37541,#4490,.T.);
#46624=EDGE_CURVE('',#37541,#37542,#30791,.T.);
#46625=EDGE_CURVE('',#37542,#37543,#4491,.T.);
#46626=EDGE_CURVE('',#37543,#37544,#20348,.T.);
#46627=EDGE_CURVE('',#37544,#37545,#30792,.T.);
#46628=EDGE_CURVE('',#37545,#37546,#20349,.T.);
#46629=EDGE_CURVE('',#37546,#37547,#4492,.T.);
#46630=EDGE_CURVE('',#37547,#37548,#30793,.T.);
#46631=EDGE_CURVE('',#37548,#37549,#4493,.T.);
#46632=EDGE_CURVE('',#37549,#37550,#20350,.T.);
#46633=EDGE_CURVE('',#37550,#37551,#30794,.T.);
#46634=EDGE_CURVE('',#37551,#37552,#20351,.T.);
#46635=EDGE_CURVE('',#37552,#36822,#4494,.T.);
#46636=EDGE_CURVE('',#37553,#37554,#30795,.T.);
#46637=EDGE_CURVE('',#37554,#36830,#20352,.T.);
#46638=EDGE_CURVE('',#37554,#37553,#30796,.T.);
#46639=EDGE_CURVE('',#37553,#37555,#20353,.T.);
#46640=EDGE_CURVE('',#37555,#37555,#30797,.T.);
#46641=EDGE_CURVE('',#37556,#37557,#30798,.T.);
#46642=EDGE_CURVE('',#37556,#37558,#20354,.T.);
#46643=EDGE_CURVE('',#37558,#37559,#30799,.T.);
#46644=EDGE_CURVE('',#37559,#37560,#20355,.T.);
#46645=EDGE_CURVE('',#37561,#37560,#30800,.T.);
#46646=EDGE_CURVE('',#37557,#37561,#30801,.T.);
#46647=EDGE_CURVE('',#37562,#37563,#30802,.T.);
#46648=EDGE_CURVE('',#37563,#37557,#20356,.T.);
#46649=EDGE_CURVE('',#37561,#37562,#20357,.T.);
#46650=EDGE_CURVE('',#37564,#37565,#30803,.T.);
#46651=EDGE_CURVE('',#37565,#37566,#20358,.T.);
#46652=EDGE_CURVE('',#37566,#37567,#30804,.T.);
#46653=EDGE_CURVE('',#37567,#37564,#20359,.T.);
#46654=EDGE_CURVE('',#37568,#37569,#30805,.T.);
#46655=EDGE_CURVE('',#37568,#37570,#20360,.T.);
#46656=EDGE_CURVE('',#37570,#37571,#30806,.T.);
#46657=EDGE_CURVE('',#37571,#37572,#20361,.T.);
#46658=EDGE_CURVE('',#37573,#37572,#30807,.T.);
#46659=EDGE_CURVE('',#37569,#37573,#30808,.T.);
#46660=EDGE_CURVE('',#37574,#37575,#30809,.T.);
#46661=EDGE_CURVE('',#37575,#37569,#20362,.T.);
#46662=EDGE_CURVE('',#37573,#37574,#20363,.T.);
#46663=EDGE_CURVE('',#37558,#37379,#30810,.T.);
#46664=EDGE_CURVE('',#37378,#37559,#30811,.T.);
#46665=EDGE_CURVE('',#37193,#37575,#338,.T.);
#46666=EDGE_CURVE('',#37574,#37194,#339,.T.);
#46667=EDGE_CURVE('',#37570,#37565,#340,.T.);
#46668=EDGE_CURVE('',#37564,#37571,#341,.T.);
#46669=EDGE_CURVE('',#37566,#37563,#342,.T.);
#46670=EDGE_CURVE('',#37562,#37567,#343,.T.);
#46671=EDGE_CURVE('',#37576,#37577,#30812,.T.);
#46672=EDGE_CURVE('',#37577,#37578,#20364,.T.);
#46673=EDGE_CURVE('',#37579,#37578,#30813,.T.);
#46674=EDGE_CURVE('',#37580,#37579,#30814,.T.);
#46675=EDGE_CURVE('',#37581,#37580,#30815,.T.);
#46676=EDGE_CURVE('',#37581,#37576,#20365,.T.);
#46677=EDGE_CURVE('',#37579,#37582,#20366,.T.);
#46678=EDGE_CURVE('',#37582,#37583,#30816,.T.);
#46679=EDGE_CURVE('',#37583,#37580,#20367,.T.);
#46680=EDGE_CURVE('',#37584,#37585,#30817,.T.);
#46681=EDGE_CURVE('',#37585,#37586,#20368,.T.);
#46682=EDGE_CURVE('',#37586,#37587,#30818,.T.);
#46683=EDGE_CURVE('',#37587,#37584,#20369,.T.);
#46684=EDGE_CURVE('',#37588,#37589,#30819,.T.);
#46685=EDGE_CURVE('',#37589,#37590,#20370,.T.);
#46686=EDGE_CURVE('',#37591,#37590,#30820,.T.);
#46687=EDGE_CURVE('',#37592,#37591,#30821,.T.);
#46688=EDGE_CURVE('',#37593,#37592,#30822,.T.);
#46689=EDGE_CURVE('',#37593,#37588,#20371,.T.);
#46690=EDGE_CURVE('',#37591,#37594,#20372,.T.);
#46691=EDGE_CURVE('',#37594,#37595,#30823,.T.);
#46692=EDGE_CURVE('',#37595,#37592,#20373,.T.);
#46693=EDGE_CURVE('',#37384,#37577,#30824,.T.);
#46694=EDGE_CURVE('',#37576,#37385,#30825,.T.);
#46695=EDGE_CURVE('',#37594,#37188,#344,.T.);
#46696=EDGE_CURVE('',#37187,#37595,#345,.T.);
#46697=EDGE_CURVE('',#37586,#37589,#346,.T.);
#46698=EDGE_CURVE('',#37588,#37587,#347,.T.);
#46699=EDGE_CURVE('',#37582,#37585,#348,.T.);
#46700=EDGE_CURVE('',#37584,#37583,#349,.T.);
#46701=EDGE_CURVE('',#37596,#37597,#30826,.T.);
#46702=EDGE_CURVE('',#37597,#37598,#20374,.T.);
#46703=EDGE_CURVE('',#37599,#37598,#30827,.T.);
#46704=EDGE_CURVE('',#37600,#37599,#30828,.T.);
#46705=EDGE_CURVE('',#37601,#37600,#30829,.T.);
#46706=EDGE_CURVE('',#37601,#37596,#20375,.T.);
#46707=EDGE_CURVE('',#37599,#37602,#20376,.T.);
#46708=EDGE_CURVE('',#37602,#37603,#30830,.T.);
#46709=EDGE_CURVE('',#37603,#37600,#20377,.T.);
#46710=EDGE_CURVE('',#37604,#37605,#30831,.T.);
#46711=EDGE_CURVE('',#37605,#37606,#20378,.T.);
#46712=EDGE_CURVE('',#37606,#37607,#30832,.T.);
#46713=EDGE_CURVE('',#37607,#37604,#20379,.T.);
#46714=EDGE_CURVE('',#37608,#37609,#30833,.T.);
#46715=EDGE_CURVE('',#37609,#37610,#20380,.T.);
#46716=EDGE_CURVE('',#37611,#37610,#30834,.T.);
#46717=EDGE_CURVE('',#37612,#37611,#30835,.T.);
#46718=EDGE_CURVE('',#37613,#37612,#30836,.T.);
#46719=EDGE_CURVE('',#37613,#37608,#20381,.T.);
#46720=EDGE_CURVE('',#37611,#37614,#20382,.T.);
#46721=EDGE_CURVE('',#37614,#37615,#30837,.T.);
#46722=EDGE_CURVE('',#37615,#37612,#20383,.T.);
#46723=EDGE_CURVE('',#37390,#37597,#30838,.T.);
#46724=EDGE_CURVE('',#37596,#37391,#30839,.T.);
#46725=EDGE_CURVE('',#37614,#37182,#350,.T.);
#46726=EDGE_CURVE('',#37181,#37615,#351,.T.);
#46727=EDGE_CURVE('',#37606,#37609,#352,.T.);
#46728=EDGE_CURVE('',#37608,#37607,#353,.T.);
#46729=EDGE_CURVE('',#37602,#37605,#354,.T.);
#46730=EDGE_CURVE('',#37604,#37603,#355,.T.);
#46731=EDGE_CURVE('',#37616,#37617,#30840,.T.);
#46732=EDGE_CURVE('',#37617,#37618,#20384,.T.);
#46733=EDGE_CURVE('',#37619,#37618,#30841,.T.);
#46734=EDGE_CURVE('',#37620,#37619,#30842,.T.);
#46735=EDGE_CURVE('',#37621,#37620,#30843,.T.);
#46736=EDGE_CURVE('',#37621,#37616,#20385,.T.);
#46737=EDGE_CURVE('',#37619,#37622,#20386,.T.);
#46738=EDGE_CURVE('',#37622,#37623,#30844,.T.);
#46739=EDGE_CURVE('',#37623,#37620,#20387,.T.);
#46740=EDGE_CURVE('',#37624,#37625,#30845,.T.);
#46741=EDGE_CURVE('',#37625,#37626,#20388,.T.);
#46742=EDGE_CURVE('',#37626,#37627,#30846,.T.);
#46743=EDGE_CURVE('',#37627,#37624,#20389,.T.);
#46744=EDGE_CURVE('',#37628,#37629,#30847,.T.);
#46745=EDGE_CURVE('',#37629,#37630,#20390,.T.);
#46746=EDGE_CURVE('',#37631,#37630,#30848,.T.);
#46747=EDGE_CURVE('',#37632,#37631,#30849,.T.);
#46748=EDGE_CURVE('',#37633,#37632,#30850,.T.);
#46749=EDGE_CURVE('',#37633,#37628,#20391,.T.);
#46750=EDGE_CURVE('',#37631,#37634,#20392,.T.);
#46751=EDGE_CURVE('',#37634,#37635,#30851,.T.);
#46752=EDGE_CURVE('',#37635,#37632,#20393,.T.);
#46753=EDGE_CURVE('',#37396,#37617,#30852,.T.);
#46754=EDGE_CURVE('',#37616,#37397,#30853,.T.);
#46755=EDGE_CURVE('',#37634,#37176,#356,.T.);
#46756=EDGE_CURVE('',#37175,#37635,#357,.T.);
#46757=EDGE_CURVE('',#37626,#37629,#358,.T.);
#46758=EDGE_CURVE('',#37628,#37627,#359,.T.);
#46759=EDGE_CURVE('',#37622,#37625,#360,.T.);
#46760=EDGE_CURVE('',#37624,#37623,#361,.T.);
#46761=EDGE_CURVE('',#37636,#37637,#30854,.T.);
#46762=EDGE_CURVE('',#37637,#37638,#20394,.T.);
#46763=EDGE_CURVE('',#37639,#37638,#30855,.T.);
#46764=EDGE_CURVE('',#37640,#37639,#30856,.T.);
#46765=EDGE_CURVE('',#37641,#37640,#30857,.T.);
#46766=EDGE_CURVE('',#37641,#37636,#20395,.T.);
#46767=EDGE_CURVE('',#37639,#37642,#20396,.T.);
#46768=EDGE_CURVE('',#37642,#37643,#30858,.T.);
#46769=EDGE_CURVE('',#37643,#37640,#20397,.T.);
#46770=EDGE_CURVE('',#37644,#37645,#30859,.T.);
#46771=EDGE_CURVE('',#37645,#37646,#20398,.T.);
#46772=EDGE_CURVE('',#37646,#37647,#30860,.T.);
#46773=EDGE_CURVE('',#37647,#37644,#20399,.T.);
#46774=EDGE_CURVE('',#37648,#37649,#30861,.T.);
#46775=EDGE_CURVE('',#37649,#37650,#20400,.T.);
#46776=EDGE_CURVE('',#37651,#37650,#30862,.T.);
#46777=EDGE_CURVE('',#37652,#37651,#30863,.T.);
#46778=EDGE_CURVE('',#37653,#37652,#30864,.T.);
#46779=EDGE_CURVE('',#37653,#37648,#20401,.T.);
#46780=EDGE_CURVE('',#37651,#37654,#20402,.T.);
#46781=EDGE_CURVE('',#37654,#37655,#30865,.T.);
#46782=EDGE_CURVE('',#37655,#37652,#20403,.T.);
#46783=EDGE_CURVE('',#37402,#37637,#30866,.T.);
#46784=EDGE_CURVE('',#37636,#37403,#30867,.T.);
#46785=EDGE_CURVE('',#37654,#37170,#362,.T.);
#46786=EDGE_CURVE('',#37169,#37655,#363,.T.);
#46787=EDGE_CURVE('',#37646,#37649,#364,.T.);
#46788=EDGE_CURVE('',#37648,#37647,#365,.T.);
#46789=EDGE_CURVE('',#37642,#37645,#366,.T.);
#46790=EDGE_CURVE('',#37644,#37643,#367,.T.);
#46791=EDGE_CURVE('',#37656,#37657,#30868,.T.);
#46792=EDGE_CURVE('',#37657,#37658,#20404,.T.);
#46793=EDGE_CURVE('',#37659,#37658,#30869,.T.);
#46794=EDGE_CURVE('',#37660,#37659,#30870,.T.);
#46795=EDGE_CURVE('',#37661,#37660,#30871,.T.);
#46796=EDGE_CURVE('',#37661,#37656,#20405,.T.);
#46797=EDGE_CURVE('',#37659,#37662,#20406,.T.);
#46798=EDGE_CURVE('',#37662,#37663,#30872,.T.);
#46799=EDGE_CURVE('',#37663,#37660,#20407,.T.);
#46800=EDGE_CURVE('',#37664,#37665,#30873,.T.);
#46801=EDGE_CURVE('',#37665,#37666,#20408,.T.);
#46802=EDGE_CURVE('',#37666,#37667,#30874,.T.);
#46803=EDGE_CURVE('',#37667,#37664,#20409,.T.);
#46804=EDGE_CURVE('',#37668,#37669,#30875,.T.);
#46805=EDGE_CURVE('',#37669,#37670,#20410,.T.);
#46806=EDGE_CURVE('',#37671,#37670,#30876,.T.);
#46807=EDGE_CURVE('',#37672,#37671,#30877,.T.);
#46808=EDGE_CURVE('',#37673,#37672,#30878,.T.);
#46809=EDGE_CURVE('',#37673,#37668,#20411,.T.);
#46810=EDGE_CURVE('',#37671,#37674,#20412,.T.);
#46811=EDGE_CURVE('',#37674,#37675,#30879,.T.);
#46812=EDGE_CURVE('',#37675,#37672,#20413,.T.);
#46813=EDGE_CURVE('',#37408,#37657,#30880,.T.);
#46814=EDGE_CURVE('',#37656,#37409,#30881,.T.);
#46815=EDGE_CURVE('',#37674,#37164,#368,.T.);
#46816=EDGE_CURVE('',#37163,#37675,#369,.T.);
#46817=EDGE_CURVE('',#37666,#37669,#370,.T.);
#46818=EDGE_CURVE('',#37668,#37667,#371,.T.);
#46819=EDGE_CURVE('',#37662,#37665,#372,.T.);
#46820=EDGE_CURVE('',#37664,#37663,#373,.T.);
#46821=EDGE_CURVE('',#37676,#37677,#30882,.T.);
#46822=EDGE_CURVE('',#37677,#37678,#20414,.T.);
#46823=EDGE_CURVE('',#37679,#37678,#30883,.T.);
#46824=EDGE_CURVE('',#37680,#37679,#30884,.T.);
#46825=EDGE_CURVE('',#37681,#37680,#30885,.T.);
#46826=EDGE_CURVE('',#37681,#37676,#20415,.T.);
#46827=EDGE_CURVE('',#37679,#37682,#20416,.T.);
#46828=EDGE_CURVE('',#37682,#37683,#30886,.T.);
#46829=EDGE_CURVE('',#37683,#37680,#20417,.T.);
#46830=EDGE_CURVE('',#37684,#37685,#30887,.T.);
#46831=EDGE_CURVE('',#37685,#37686,#20418,.T.);
#46832=EDGE_CURVE('',#37686,#37687,#30888,.T.);
#46833=EDGE_CURVE('',#37687,#37684,#20419,.T.);
#46834=EDGE_CURVE('',#37688,#37689,#30889,.T.);
#46835=EDGE_CURVE('',#37689,#37690,#20420,.T.);
#46836=EDGE_CURVE('',#37691,#37690,#30890,.T.);
#46837=EDGE_CURVE('',#37692,#37691,#30891,.T.);
#46838=EDGE_CURVE('',#37693,#37692,#30892,.T.);
#46839=EDGE_CURVE('',#37693,#37688,#20421,.T.);
#46840=EDGE_CURVE('',#37691,#37694,#20422,.T.);
#46841=EDGE_CURVE('',#37694,#37695,#30893,.T.);
#46842=EDGE_CURVE('',#37695,#37692,#20423,.T.);
#46843=EDGE_CURVE('',#37414,#37677,#30894,.T.);
#46844=EDGE_CURVE('',#37676,#37415,#30895,.T.);
#46845=EDGE_CURVE('',#37694,#37158,#374,.T.);
#46846=EDGE_CURVE('',#37157,#37695,#375,.T.);
#46847=EDGE_CURVE('',#37686,#37689,#376,.T.);
#46848=EDGE_CURVE('',#37688,#37687,#377,.T.);
#46849=EDGE_CURVE('',#37682,#37685,#378,.T.);
#46850=EDGE_CURVE('',#37684,#37683,#379,.T.);
#46851=EDGE_CURVE('',#37696,#37697,#30896,.T.);
#46852=EDGE_CURVE('',#37697,#37698,#20424,.T.);
#46853=EDGE_CURVE('',#37699,#37698,#30897,.T.);
#46854=EDGE_CURVE('',#37700,#37699,#30898,.T.);
#46855=EDGE_CURVE('',#37701,#37700,#30899,.T.);
#46856=EDGE_CURVE('',#37701,#37696,#20425,.T.);
#46857=EDGE_CURVE('',#37699,#37702,#20426,.T.);
#46858=EDGE_CURVE('',#37702,#37703,#30900,.T.);
#46859=EDGE_CURVE('',#37703,#37700,#20427,.T.);
#46860=EDGE_CURVE('',#37704,#37705,#30901,.T.);
#46861=EDGE_CURVE('',#37705,#37706,#20428,.T.);
#46862=EDGE_CURVE('',#37706,#37707,#30902,.T.);
#46863=EDGE_CURVE('',#37707,#37704,#20429,.T.);
#46864=EDGE_CURVE('',#37708,#37709,#30903,.T.);
#46865=EDGE_CURVE('',#37709,#37710,#20430,.T.);
#46866=EDGE_CURVE('',#37711,#37710,#30904,.T.);
#46867=EDGE_CURVE('',#37712,#37711,#30905,.T.);
#46868=EDGE_CURVE('',#37713,#37712,#30906,.T.);
#46869=EDGE_CURVE('',#37713,#37708,#20431,.T.);
#46870=EDGE_CURVE('',#37711,#37714,#20432,.T.);
#46871=EDGE_CURVE('',#37714,#37715,#30907,.T.);
#46872=EDGE_CURVE('',#37715,#37712,#20433,.T.);
#46873=EDGE_CURVE('',#37420,#37697,#30908,.T.);
#46874=EDGE_CURVE('',#37696,#37421,#30909,.T.);
#46875=EDGE_CURVE('',#37714,#37152,#380,.T.);
#46876=EDGE_CURVE('',#37151,#37715,#381,.T.);
#46877=EDGE_CURVE('',#37706,#37709,#382,.T.);
#46878=EDGE_CURVE('',#37708,#37707,#383,.T.);
#46879=EDGE_CURVE('',#37702,#37705,#384,.T.);
#46880=EDGE_CURVE('',#37704,#37703,#385,.T.);
#46881=EDGE_CURVE('',#37716,#37717,#30910,.T.);
#46882=EDGE_CURVE('',#37717,#37718,#20434,.T.);
#46883=EDGE_CURVE('',#37719,#37718,#30911,.T.);
#46884=EDGE_CURVE('',#37720,#37719,#30912,.T.);
#46885=EDGE_CURVE('',#37721,#37720,#30913,.T.);
#46886=EDGE_CURVE('',#37721,#37716,#20435,.T.);
#46887=EDGE_CURVE('',#37719,#37722,#20436,.T.);
#46888=EDGE_CURVE('',#37722,#37723,#30914,.T.);
#46889=EDGE_CURVE('',#37723,#37720,#20437,.T.);
#46890=EDGE_CURVE('',#37724,#37725,#30915,.T.);
#46891=EDGE_CURVE('',#37725,#37726,#20438,.T.);
#46892=EDGE_CURVE('',#37726,#37727,#30916,.T.);
#46893=EDGE_CURVE('',#37727,#37724,#20439,.T.);
#46894=EDGE_CURVE('',#37728,#37729,#30917,.T.);
#46895=EDGE_CURVE('',#37729,#37730,#20440,.T.);
#46896=EDGE_CURVE('',#37731,#37730,#30918,.T.);
#46897=EDGE_CURVE('',#37732,#37731,#30919,.T.);
#46898=EDGE_CURVE('',#37733,#37732,#30920,.T.);
#46899=EDGE_CURVE('',#37733,#37728,#20441,.T.);
#46900=EDGE_CURVE('',#37731,#37734,#20442,.T.);
#46901=EDGE_CURVE('',#37734,#37735,#30921,.T.);
#46902=EDGE_CURVE('',#37735,#37732,#20443,.T.);
#46903=EDGE_CURVE('',#37426,#37717,#30922,.T.);
#46904=EDGE_CURVE('',#37716,#37427,#30923,.T.);
#46905=EDGE_CURVE('',#37734,#37146,#386,.T.);
#46906=EDGE_CURVE('',#37145,#37735,#387,.T.);
#46907=EDGE_CURVE('',#37726,#37729,#388,.T.);
#46908=EDGE_CURVE('',#37728,#37727,#389,.T.);
#46909=EDGE_CURVE('',#37722,#37725,#390,.T.);
#46910=EDGE_CURVE('',#37724,#37723,#391,.T.);
#46911=EDGE_CURVE('',#37736,#37737,#30924,.T.);
#46912=EDGE_CURVE('',#37737,#37738,#20444,.T.);
#46913=EDGE_CURVE('',#37739,#37738,#30925,.T.);
#46914=EDGE_CURVE('',#37740,#37739,#30926,.T.);
#46915=EDGE_CURVE('',#37741,#37740,#30927,.T.);
#46916=EDGE_CURVE('',#37741,#37736,#20445,.T.);
#46917=EDGE_CURVE('',#37739,#37742,#20446,.T.);
#46918=EDGE_CURVE('',#37742,#37743,#30928,.T.);
#46919=EDGE_CURVE('',#37743,#37740,#20447,.T.);
#46920=EDGE_CURVE('',#37744,#37745,#30929,.T.);
#46921=EDGE_CURVE('',#37745,#37746,#20448,.T.);
#46922=EDGE_CURVE('',#37746,#37747,#30930,.T.);
#46923=EDGE_CURVE('',#37747,#37744,#20449,.T.);
#46924=EDGE_CURVE('',#37748,#37749,#30931,.T.);
#46925=EDGE_CURVE('',#37749,#37750,#20450,.T.);
#46926=EDGE_CURVE('',#37751,#37750,#30932,.T.);
#46927=EDGE_CURVE('',#37752,#37751,#30933,.T.);
#46928=EDGE_CURVE('',#37753,#37752,#30934,.T.);
#46929=EDGE_CURVE('',#37753,#37748,#20451,.T.);
#46930=EDGE_CURVE('',#37751,#37754,#20452,.T.);
#46931=EDGE_CURVE('',#37754,#37755,#30935,.T.);
#46932=EDGE_CURVE('',#37755,#37752,#20453,.T.);
#46933=EDGE_CURVE('',#37432,#37737,#30936,.T.);
#46934=EDGE_CURVE('',#37736,#37433,#30937,.T.);
#46935=EDGE_CURVE('',#37754,#37140,#392,.T.);
#46936=EDGE_CURVE('',#37139,#37755,#393,.T.);
#46937=EDGE_CURVE('',#37746,#37749,#394,.T.);
#46938=EDGE_CURVE('',#37748,#37747,#395,.T.);
#46939=EDGE_CURVE('',#37742,#37745,#396,.T.);
#46940=EDGE_CURVE('',#37744,#37743,#397,.T.);
#46941=EDGE_CURVE('',#37756,#37757,#30938,.T.);
#46942=EDGE_CURVE('',#37757,#37758,#20454,.T.);
#46943=EDGE_CURVE('',#37759,#37758,#30939,.T.);
#46944=EDGE_CURVE('',#37760,#37759,#30940,.T.);
#46945=EDGE_CURVE('',#37761,#37760,#30941,.T.);
#46946=EDGE_CURVE('',#37761,#37756,#20455,.T.);
#46947=EDGE_CURVE('',#37759,#37762,#20456,.T.);
#46948=EDGE_CURVE('',#37762,#37763,#30942,.T.);
#46949=EDGE_CURVE('',#37763,#37760,#20457,.T.);
#46950=EDGE_CURVE('',#37764,#37765,#30943,.T.);
#46951=EDGE_CURVE('',#37765,#37766,#20458,.T.);
#46952=EDGE_CURVE('',#37766,#37767,#30944,.T.);
#46953=EDGE_CURVE('',#37767,#37764,#20459,.T.);
#46954=EDGE_CURVE('',#37768,#37769,#30945,.T.);
#46955=EDGE_CURVE('',#37769,#37770,#20460,.T.);
#46956=EDGE_CURVE('',#37771,#37770,#30946,.T.);
#46957=EDGE_CURVE('',#37772,#37771,#30947,.T.);
#46958=EDGE_CURVE('',#37773,#37772,#30948,.T.);
#46959=EDGE_CURVE('',#37773,#37768,#20461,.T.);
#46960=EDGE_CURVE('',#37771,#37774,#20462,.T.);
#46961=EDGE_CURVE('',#37774,#37775,#30949,.T.);
#46962=EDGE_CURVE('',#37775,#37772,#20463,.T.);
#46963=EDGE_CURVE('',#37438,#37757,#30950,.T.);
#46964=EDGE_CURVE('',#37756,#37439,#30951,.T.);
#46965=EDGE_CURVE('',#37774,#37134,#398,.T.);
#46966=EDGE_CURVE('',#37133,#37775,#399,.T.);
#46967=EDGE_CURVE('',#37766,#37769,#400,.T.);
#46968=EDGE_CURVE('',#37768,#37767,#401,.T.);
#46969=EDGE_CURVE('',#37762,#37765,#402,.T.);
#46970=EDGE_CURVE('',#37764,#37763,#403,.T.);
#46971=EDGE_CURVE('',#37776,#37777,#30952,.T.);
#46972=EDGE_CURVE('',#37777,#37778,#20464,.T.);
#46973=EDGE_CURVE('',#37779,#37778,#30953,.T.);
#46974=EDGE_CURVE('',#37780,#37779,#30954,.T.);
#46975=EDGE_CURVE('',#37781,#37780,#30955,.T.);
#46976=EDGE_CURVE('',#37781,#37776,#20465,.T.);
#46977=EDGE_CURVE('',#37779,#37782,#20466,.T.);
#46978=EDGE_CURVE('',#37782,#37783,#30956,.T.);
#46979=EDGE_CURVE('',#37783,#37780,#20467,.T.);
#46980=EDGE_CURVE('',#37784,#37785,#30957,.T.);
#46981=EDGE_CURVE('',#37785,#37786,#20468,.T.);
#46982=EDGE_CURVE('',#37786,#37787,#30958,.T.);
#46983=EDGE_CURVE('',#37787,#37784,#20469,.T.);
#46984=EDGE_CURVE('',#37788,#37789,#30959,.T.);
#46985=EDGE_CURVE('',#37789,#37790,#20470,.T.);
#46986=EDGE_CURVE('',#37791,#37790,#30960,.T.);
#46987=EDGE_CURVE('',#37792,#37791,#30961,.T.);
#46988=EDGE_CURVE('',#37793,#37792,#30962,.T.);
#46989=EDGE_CURVE('',#37793,#37788,#20471,.T.);
#46990=EDGE_CURVE('',#37791,#37794,#20472,.T.);
#46991=EDGE_CURVE('',#37794,#37795,#30963,.T.);
#46992=EDGE_CURVE('',#37795,#37792,#20473,.T.);
#46993=EDGE_CURVE('',#37444,#37777,#30964,.T.);
#46994=EDGE_CURVE('',#37776,#37445,#30965,.T.);
#46995=EDGE_CURVE('',#37794,#37128,#404,.T.);
#46996=EDGE_CURVE('',#37127,#37795,#405,.T.);
#46997=EDGE_CURVE('',#37786,#37789,#406,.T.);
#46998=EDGE_CURVE('',#37788,#37787,#407,.T.);
#46999=EDGE_CURVE('',#37782,#37785,#408,.T.);
#47000=EDGE_CURVE('',#37784,#37783,#409,.T.);
#47001=EDGE_CURVE('',#37796,#37797,#30966,.T.);
#47002=EDGE_CURVE('',#37797,#37798,#20474,.T.);
#47003=EDGE_CURVE('',#37799,#37798,#30967,.T.);
#47004=EDGE_CURVE('',#37800,#37799,#30968,.T.);
#47005=EDGE_CURVE('',#37801,#37800,#30969,.T.);
#47006=EDGE_CURVE('',#37801,#37796,#20475,.T.);
#47007=EDGE_CURVE('',#37799,#37802,#20476,.T.);
#47008=EDGE_CURVE('',#37802,#37803,#30970,.T.);
#47009=EDGE_CURVE('',#37803,#37800,#20477,.T.);
#47010=EDGE_CURVE('',#37804,#37805,#30971,.T.);
#47011=EDGE_CURVE('',#37805,#37806,#20478,.T.);
#47012=EDGE_CURVE('',#37806,#37807,#30972,.T.);
#47013=EDGE_CURVE('',#37807,#37804,#20479,.T.);
#47014=EDGE_CURVE('',#37808,#37809,#30973,.T.);
#47015=EDGE_CURVE('',#37809,#37810,#20480,.T.);
#47016=EDGE_CURVE('',#37811,#37810,#30974,.T.);
#47017=EDGE_CURVE('',#37812,#37811,#30975,.T.);
#47018=EDGE_CURVE('',#37813,#37812,#30976,.T.);
#47019=EDGE_CURVE('',#37813,#37808,#20481,.T.);
#47020=EDGE_CURVE('',#37811,#37814,#20482,.T.);
#47021=EDGE_CURVE('',#37814,#37815,#30977,.T.);
#47022=EDGE_CURVE('',#37815,#37812,#20483,.T.);
#47023=EDGE_CURVE('',#37450,#37797,#30978,.T.);
#47024=EDGE_CURVE('',#37796,#37451,#30979,.T.);
#47025=EDGE_CURVE('',#37814,#37122,#410,.T.);
#47026=EDGE_CURVE('',#37121,#37815,#411,.T.);
#47027=EDGE_CURVE('',#37806,#37809,#412,.T.);
#47028=EDGE_CURVE('',#37808,#37807,#413,.T.);
#47029=EDGE_CURVE('',#37802,#37805,#414,.T.);
#47030=EDGE_CURVE('',#37804,#37803,#415,.T.);
#47031=EDGE_CURVE('',#37816,#37817,#30980,.T.);
#47032=EDGE_CURVE('',#37817,#37818,#20484,.T.);
#47033=EDGE_CURVE('',#37819,#37818,#30981,.T.);
#47034=EDGE_CURVE('',#37820,#37819,#30982,.T.);
#47035=EDGE_CURVE('',#37821,#37820,#30983,.T.);
#47036=EDGE_CURVE('',#37821,#37816,#20485,.T.);
#47037=EDGE_CURVE('',#37819,#37822,#20486,.T.);
#47038=EDGE_CURVE('',#37822,#37823,#30984,.T.);
#47039=EDGE_CURVE('',#37823,#37820,#20487,.T.);
#47040=EDGE_CURVE('',#37824,#37825,#30985,.T.);
#47041=EDGE_CURVE('',#37825,#37826,#20488,.T.);
#47042=EDGE_CURVE('',#37826,#37827,#30986,.T.);
#47043=EDGE_CURVE('',#37827,#37824,#20489,.T.);
#47044=EDGE_CURVE('',#37828,#37829,#30987,.T.);
#47045=EDGE_CURVE('',#37829,#37830,#20490,.T.);
#47046=EDGE_CURVE('',#37831,#37830,#30988,.T.);
#47047=EDGE_CURVE('',#37832,#37831,#30989,.T.);
#47048=EDGE_CURVE('',#37833,#37832,#30990,.T.);
#47049=EDGE_CURVE('',#37833,#37828,#20491,.T.);
#47050=EDGE_CURVE('',#37831,#37834,#20492,.T.);
#47051=EDGE_CURVE('',#37834,#37835,#30991,.T.);
#47052=EDGE_CURVE('',#37835,#37832,#20493,.T.);
#47053=EDGE_CURVE('',#37456,#37817,#30992,.T.);
#47054=EDGE_CURVE('',#37816,#37457,#30993,.T.);
#47055=EDGE_CURVE('',#37834,#37116,#416,.T.);
#47056=EDGE_CURVE('',#37115,#37835,#417,.T.);
#47057=EDGE_CURVE('',#37826,#37829,#418,.T.);
#47058=EDGE_CURVE('',#37828,#37827,#419,.T.);
#47059=EDGE_CURVE('',#37822,#37825,#420,.T.);
#47060=EDGE_CURVE('',#37824,#37823,#421,.T.);
#47061=EDGE_CURVE('',#37836,#37837,#30994,.T.);
#47062=EDGE_CURVE('',#37837,#37838,#20494,.T.);
#47063=EDGE_CURVE('',#37839,#37838,#30995,.T.);
#47064=EDGE_CURVE('',#37840,#37839,#30996,.T.);
#47065=EDGE_CURVE('',#37841,#37840,#30997,.T.);
#47066=EDGE_CURVE('',#37841,#37836,#20495,.T.);
#47067=EDGE_CURVE('',#37839,#37842,#20496,.T.);
#47068=EDGE_CURVE('',#37842,#37843,#30998,.T.);
#47069=EDGE_CURVE('',#37843,#37840,#20497,.T.);
#47070=EDGE_CURVE('',#37844,#37845,#30999,.T.);
#47071=EDGE_CURVE('',#37845,#37846,#20498,.T.);
#47072=EDGE_CURVE('',#37846,#37847,#31000,.T.);
#47073=EDGE_CURVE('',#37847,#37844,#20499,.T.);
#47074=EDGE_CURVE('',#37848,#37849,#31001,.T.);
#47075=EDGE_CURVE('',#37849,#37850,#20500,.T.);
#47076=EDGE_CURVE('',#37851,#37850,#31002,.T.);
#47077=EDGE_CURVE('',#37852,#37851,#31003,.T.);
#47078=EDGE_CURVE('',#37853,#37852,#31004,.T.);
#47079=EDGE_CURVE('',#37853,#37848,#20501,.T.);
#47080=EDGE_CURVE('',#37851,#37854,#20502,.T.);
#47081=EDGE_CURVE('',#37854,#37855,#31005,.T.);
#47082=EDGE_CURVE('',#37855,#37852,#20503,.T.);
#47083=EDGE_CURVE('',#37462,#37837,#31006,.T.);
#47084=EDGE_CURVE('',#37836,#37463,#31007,.T.);
#47085=EDGE_CURVE('',#37854,#37110,#422,.T.);
#47086=EDGE_CURVE('',#37109,#37855,#423,.T.);
#47087=EDGE_CURVE('',#37846,#37849,#424,.T.);
#47088=EDGE_CURVE('',#37848,#37847,#425,.T.);
#47089=EDGE_CURVE('',#37842,#37845,#426,.T.);
#47090=EDGE_CURVE('',#37844,#37843,#427,.T.);
#47091=EDGE_CURVE('',#37856,#37857,#31008,.T.);
#47092=EDGE_CURVE('',#37857,#37858,#20504,.T.);
#47093=EDGE_CURVE('',#37859,#37858,#31009,.T.);
#47094=EDGE_CURVE('',#37860,#37859,#31010,.T.);
#47095=EDGE_CURVE('',#37861,#37860,#31011,.T.);
#47096=EDGE_CURVE('',#37861,#37856,#20505,.T.);
#47097=EDGE_CURVE('',#37859,#37862,#20506,.T.);
#47098=EDGE_CURVE('',#37862,#37863,#31012,.T.);
#47099=EDGE_CURVE('',#37863,#37860,#20507,.T.);
#47100=EDGE_CURVE('',#37864,#37865,#31013,.T.);
#47101=EDGE_CURVE('',#37865,#37866,#20508,.T.);
#47102=EDGE_CURVE('',#37866,#37867,#31014,.T.);
#47103=EDGE_CURVE('',#37867,#37864,#20509,.T.);
#47104=EDGE_CURVE('',#37868,#37869,#31015,.T.);
#47105=EDGE_CURVE('',#37869,#37870,#20510,.T.);
#47106=EDGE_CURVE('',#37871,#37870,#31016,.T.);
#47107=EDGE_CURVE('',#37872,#37871,#31017,.T.);
#47108=EDGE_CURVE('',#37873,#37872,#31018,.T.);
#47109=EDGE_CURVE('',#37873,#37868,#20511,.T.);
#47110=EDGE_CURVE('',#37871,#37874,#20512,.T.);
#47111=EDGE_CURVE('',#37874,#37875,#31019,.T.);
#47112=EDGE_CURVE('',#37875,#37872,#20513,.T.);
#47113=EDGE_CURVE('',#37466,#37857,#31020,.T.);
#47114=EDGE_CURVE('',#37856,#37467,#31021,.T.);
#47115=EDGE_CURVE('',#37874,#37106,#428,.T.);
#47116=EDGE_CURVE('',#37105,#37875,#429,.T.);
#47117=EDGE_CURVE('',#37866,#37869,#430,.T.);
#47118=EDGE_CURVE('',#37868,#37867,#431,.T.);
#47119=EDGE_CURVE('',#37862,#37865,#432,.T.);
#47120=EDGE_CURVE('',#37864,#37863,#433,.T.);
#47121=EDGE_CURVE('',#37876,#37877,#31022,.T.);
#47122=EDGE_CURVE('',#37877,#37878,#20514,.T.);
#47123=EDGE_CURVE('',#37879,#37878,#31023,.T.);
#47124=EDGE_CURVE('',#37880,#37879,#31024,.T.);
#47125=EDGE_CURVE('',#37881,#37880,#31025,.T.);
#47126=EDGE_CURVE('',#37881,#37876,#20515,.T.);
#47127=EDGE_CURVE('',#37879,#37882,#20516,.T.);
#47128=EDGE_CURVE('',#37882,#37883,#31026,.T.);
#47129=EDGE_CURVE('',#37883,#37880,#20517,.T.);
#47130=EDGE_CURVE('',#37884,#37885,#31027,.T.);
#47131=EDGE_CURVE('',#37885,#37886,#20518,.T.);
#47132=EDGE_CURVE('',#37886,#37887,#31028,.T.);
#47133=EDGE_CURVE('',#37887,#37884,#20519,.T.);
#47134=EDGE_CURVE('',#37888,#37889,#31029,.T.);
#47135=EDGE_CURVE('',#37889,#37890,#20520,.T.);
#47136=EDGE_CURVE('',#37891,#37890,#31030,.T.);
#47137=EDGE_CURVE('',#37892,#37891,#31031,.T.);
#47138=EDGE_CURVE('',#37893,#37892,#31032,.T.);
#47139=EDGE_CURVE('',#37893,#37888,#20521,.T.);
#47140=EDGE_CURVE('',#37891,#37894,#20522,.T.);
#47141=EDGE_CURVE('',#37894,#37895,#31033,.T.);
#47142=EDGE_CURVE('',#37895,#37892,#20523,.T.);
#47143=EDGE_CURVE('',#37472,#37877,#31034,.T.);
#47144=EDGE_CURVE('',#37876,#37473,#31035,.T.);
#47145=EDGE_CURVE('',#37894,#37100,#434,.T.);
#47146=EDGE_CURVE('',#37099,#37895,#435,.T.);
#47147=EDGE_CURVE('',#37886,#37889,#436,.T.);
#47148=EDGE_CURVE('',#37888,#37887,#437,.T.);
#47149=EDGE_CURVE('',#37882,#37885,#438,.T.);
#47150=EDGE_CURVE('',#37884,#37883,#439,.T.);
#47151=EDGE_CURVE('',#37896,#37897,#31036,.T.);
#47152=EDGE_CURVE('',#37897,#37898,#20524,.T.);
#47153=EDGE_CURVE('',#37899,#37898,#31037,.T.);
#47154=EDGE_CURVE('',#37900,#37899,#31038,.T.);
#47155=EDGE_CURVE('',#37901,#37900,#31039,.T.);
#47156=EDGE_CURVE('',#37901,#37896,#20525,.T.);
#47157=EDGE_CURVE('',#37899,#37902,#20526,.T.);
#47158=EDGE_CURVE('',#37902,#37903,#31040,.T.);
#47159=EDGE_CURVE('',#37903,#37900,#20527,.T.);
#47160=EDGE_CURVE('',#37904,#37905,#31041,.T.);
#47161=EDGE_CURVE('',#37905,#37906,#20528,.T.);
#47162=EDGE_CURVE('',#37906,#37907,#31042,.T.);
#47163=EDGE_CURVE('',#37907,#37904,#20529,.T.);
#47164=EDGE_CURVE('',#37908,#37909,#31043,.T.);
#47165=EDGE_CURVE('',#37909,#37910,#20530,.T.);
#47166=EDGE_CURVE('',#37911,#37910,#31044,.T.);
#47167=EDGE_CURVE('',#37912,#37911,#31045,.T.);
#47168=EDGE_CURVE('',#37913,#37912,#31046,.T.);
#47169=EDGE_CURVE('',#37913,#37908,#20531,.T.);
#47170=EDGE_CURVE('',#37911,#37914,#20532,.T.);
#47171=EDGE_CURVE('',#37914,#37915,#31047,.T.);
#47172=EDGE_CURVE('',#37915,#37912,#20533,.T.);
#47173=EDGE_CURVE('',#37478,#37897,#31048,.T.);
#47174=EDGE_CURVE('',#37896,#37479,#31049,.T.);
#47175=EDGE_CURVE('',#37914,#37094,#440,.T.);
#47176=EDGE_CURVE('',#37093,#37915,#441,.T.);
#47177=EDGE_CURVE('',#37906,#37909,#442,.T.);
#47178=EDGE_CURVE('',#37908,#37907,#443,.T.);
#47179=EDGE_CURVE('',#37902,#37905,#444,.T.);
#47180=EDGE_CURVE('',#37904,#37903,#445,.T.);
#47181=EDGE_CURVE('',#37916,#37917,#31050,.T.);
#47182=EDGE_CURVE('',#37917,#37918,#20534,.T.);
#47183=EDGE_CURVE('',#37919,#37918,#31051,.T.);
#47184=EDGE_CURVE('',#37920,#37919,#31052,.T.);
#47185=EDGE_CURVE('',#37921,#37920,#31053,.T.);
#47186=EDGE_CURVE('',#37921,#37916,#20535,.T.);
#47187=EDGE_CURVE('',#37919,#37922,#20536,.T.);
#47188=EDGE_CURVE('',#37922,#37923,#31054,.T.);
#47189=EDGE_CURVE('',#37923,#37920,#20537,.T.);
#47190=EDGE_CURVE('',#37924,#37925,#31055,.T.);
#47191=EDGE_CURVE('',#37925,#37926,#20538,.T.);
#47192=EDGE_CURVE('',#37926,#37927,#31056,.T.);
#47193=EDGE_CURVE('',#37927,#37924,#20539,.T.);
#47194=EDGE_CURVE('',#37928,#37929,#31057,.T.);
#47195=EDGE_CURVE('',#37929,#37930,#20540,.T.);
#47196=EDGE_CURVE('',#37931,#37930,#31058,.T.);
#47197=EDGE_CURVE('',#37932,#37931,#31059,.T.);
#47198=EDGE_CURVE('',#37933,#37932,#31060,.T.);
#47199=EDGE_CURVE('',#37933,#37928,#20541,.T.);
#47200=EDGE_CURVE('',#37931,#37934,#20542,.T.);
#47201=EDGE_CURVE('',#37934,#37935,#31061,.T.);
#47202=EDGE_CURVE('',#37935,#37932,#20543,.T.);
#47203=EDGE_CURVE('',#37484,#37917,#31062,.T.);
#47204=EDGE_CURVE('',#37916,#37485,#31063,.T.);
#47205=EDGE_CURVE('',#37934,#37088,#446,.T.);
#47206=EDGE_CURVE('',#37087,#37935,#447,.T.);
#47207=EDGE_CURVE('',#37926,#37929,#448,.T.);
#47208=EDGE_CURVE('',#37928,#37927,#449,.T.);
#47209=EDGE_CURVE('',#37922,#37925,#450,.T.);
#47210=EDGE_CURVE('',#37924,#37923,#451,.T.);
#47211=EDGE_CURVE('',#37936,#37937,#31064,.T.);
#47212=EDGE_CURVE('',#37937,#37938,#20544,.T.);
#47213=EDGE_CURVE('',#37939,#37938,#31065,.T.);
#47214=EDGE_CURVE('',#37940,#37939,#31066,.T.);
#47215=EDGE_CURVE('',#37941,#37940,#31067,.T.);
#47216=EDGE_CURVE('',#37941,#37936,#20545,.T.);
#47217=EDGE_CURVE('',#37939,#37942,#20546,.T.);
#47218=EDGE_CURVE('',#37942,#37943,#31068,.T.);
#47219=EDGE_CURVE('',#37943,#37940,#20547,.T.);
#47220=EDGE_CURVE('',#37944,#37945,#31069,.T.);
#47221=EDGE_CURVE('',#37945,#37946,#20548,.T.);
#47222=EDGE_CURVE('',#37946,#37947,#31070,.T.);
#47223=EDGE_CURVE('',#37947,#37944,#20549,.T.);
#47224=EDGE_CURVE('',#37948,#37949,#31071,.T.);
#47225=EDGE_CURVE('',#37949,#37950,#20550,.T.);
#47226=EDGE_CURVE('',#37951,#37950,#31072,.T.);
#47227=EDGE_CURVE('',#37952,#37951,#31073,.T.);
#47228=EDGE_CURVE('',#37953,#37952,#31074,.T.);
#47229=EDGE_CURVE('',#37953,#37948,#20551,.T.);
#47230=EDGE_CURVE('',#37951,#37954,#20552,.T.);
#47231=EDGE_CURVE('',#37954,#37955,#31075,.T.);
#47232=EDGE_CURVE('',#37955,#37952,#20553,.T.);
#47233=EDGE_CURVE('',#37490,#37937,#31076,.T.);
#47234=EDGE_CURVE('',#37936,#37491,#31077,.T.);
#47235=EDGE_CURVE('',#37954,#37082,#452,.T.);
#47236=EDGE_CURVE('',#37081,#37955,#453,.T.);
#47237=EDGE_CURVE('',#37946,#37949,#454,.T.);
#47238=EDGE_CURVE('',#37948,#37947,#455,.T.);
#47239=EDGE_CURVE('',#37942,#37945,#456,.T.);
#47240=EDGE_CURVE('',#37944,#37943,#457,.T.);
#47241=EDGE_CURVE('',#37956,#37957,#31078,.T.);
#47242=EDGE_CURVE('',#37957,#37958,#20554,.T.);
#47243=EDGE_CURVE('',#37959,#37958,#31079,.T.);
#47244=EDGE_CURVE('',#37960,#37959,#31080,.T.);
#47245=EDGE_CURVE('',#37961,#37960,#31081,.T.);
#47246=EDGE_CURVE('',#37961,#37956,#20555,.T.);
#47247=EDGE_CURVE('',#37959,#37962,#20556,.T.);
#47248=EDGE_CURVE('',#37962,#37963,#31082,.T.);
#47249=EDGE_CURVE('',#37963,#37960,#20557,.T.);
#47250=EDGE_CURVE('',#37964,#37965,#31083,.T.);
#47251=EDGE_CURVE('',#37965,#37966,#20558,.T.);
#47252=EDGE_CURVE('',#37966,#37967,#31084,.T.);
#47253=EDGE_CURVE('',#37967,#37964,#20559,.T.);
#47254=EDGE_CURVE('',#37968,#37969,#31085,.T.);
#47255=EDGE_CURVE('',#37969,#37970,#20560,.T.);
#47256=EDGE_CURVE('',#37971,#37970,#31086,.T.);
#47257=EDGE_CURVE('',#37972,#37971,#31087,.T.);
#47258=EDGE_CURVE('',#37973,#37972,#31088,.T.);
#47259=EDGE_CURVE('',#37973,#37968,#20561,.T.);
#47260=EDGE_CURVE('',#37971,#37974,#20562,.T.);
#47261=EDGE_CURVE('',#37974,#37975,#31089,.T.);
#47262=EDGE_CURVE('',#37975,#37972,#20563,.T.);
#47263=EDGE_CURVE('',#37496,#37957,#31090,.T.);
#47264=EDGE_CURVE('',#37956,#37497,#31091,.T.);
#47265=EDGE_CURVE('',#37974,#37076,#458,.T.);
#47266=EDGE_CURVE('',#37075,#37975,#459,.T.);
#47267=EDGE_CURVE('',#37966,#37969,#460,.T.);
#47268=EDGE_CURVE('',#37968,#37967,#461,.T.);
#47269=EDGE_CURVE('',#37962,#37965,#462,.T.);
#47270=EDGE_CURVE('',#37964,#37963,#463,.T.);
#47271=EDGE_CURVE('',#37976,#37977,#31092,.T.);
#47272=EDGE_CURVE('',#37977,#37978,#20564,.T.);
#47273=EDGE_CURVE('',#37979,#37978,#31093,.T.);
#47274=EDGE_CURVE('',#37980,#37979,#31094,.T.);
#47275=EDGE_CURVE('',#37981,#37980,#31095,.T.);
#47276=EDGE_CURVE('',#37981,#37976,#20565,.T.);
#47277=EDGE_CURVE('',#37979,#37982,#20566,.T.);
#47278=EDGE_CURVE('',#37982,#37983,#31096,.T.);
#47279=EDGE_CURVE('',#37983,#37980,#20567,.T.);
#47280=EDGE_CURVE('',#37984,#37985,#31097,.T.);
#47281=EDGE_CURVE('',#37985,#37986,#20568,.T.);
#47282=EDGE_CURVE('',#37986,#37987,#31098,.T.);
#47283=EDGE_CURVE('',#37987,#37984,#20569,.T.);
#47284=EDGE_CURVE('',#37988,#37989,#31099,.T.);
#47285=EDGE_CURVE('',#37989,#37990,#20570,.T.);
#47286=EDGE_CURVE('',#37991,#37990,#31100,.T.);
#47287=EDGE_CURVE('',#37992,#37991,#31101,.T.);
#47288=EDGE_CURVE('',#37993,#37992,#31102,.T.);
#47289=EDGE_CURVE('',#37993,#37988,#20571,.T.);
#47290=EDGE_CURVE('',#37991,#37994,#20572,.T.);
#47291=EDGE_CURVE('',#37994,#37995,#31103,.T.);
#47292=EDGE_CURVE('',#37995,#37992,#20573,.T.);
#47293=EDGE_CURVE('',#37502,#37977,#31104,.T.);
#47294=EDGE_CURVE('',#37976,#37503,#31105,.T.);
#47295=EDGE_CURVE('',#37994,#37070,#464,.T.);
#47296=EDGE_CURVE('',#37069,#37995,#465,.T.);
#47297=EDGE_CURVE('',#37986,#37989,#466,.T.);
#47298=EDGE_CURVE('',#37988,#37987,#467,.T.);
#47299=EDGE_CURVE('',#37982,#37985,#468,.T.);
#47300=EDGE_CURVE('',#37984,#37983,#469,.T.);
#47301=EDGE_CURVE('',#37996,#37997,#31106,.T.);
#47302=EDGE_CURVE('',#37997,#37998,#20574,.T.);
#47303=EDGE_CURVE('',#37999,#37998,#31107,.T.);
#47304=EDGE_CURVE('',#38000,#37999,#31108,.T.);
#47305=EDGE_CURVE('',#38001,#38000,#31109,.T.);
#47306=EDGE_CURVE('',#38001,#37996,#20575,.T.);
#47307=EDGE_CURVE('',#37999,#38002,#20576,.T.);
#47308=EDGE_CURVE('',#38002,#38003,#31110,.T.);
#47309=EDGE_CURVE('',#38003,#38000,#20577,.T.);
#47310=EDGE_CURVE('',#38004,#38005,#31111,.T.);
#47311=EDGE_CURVE('',#38005,#38006,#20578,.T.);
#47312=EDGE_CURVE('',#38006,#38007,#31112,.T.);
#47313=EDGE_CURVE('',#38007,#38004,#20579,.T.);
#47314=EDGE_CURVE('',#38008,#38009,#31113,.T.);
#47315=EDGE_CURVE('',#38009,#38010,#20580,.T.);
#47316=EDGE_CURVE('',#38011,#38010,#31114,.T.);
#47317=EDGE_CURVE('',#38012,#38011,#31115,.T.);
#47318=EDGE_CURVE('',#38013,#38012,#31116,.T.);
#47319=EDGE_CURVE('',#38013,#38008,#20581,.T.);
#47320=EDGE_CURVE('',#38011,#38014,#20582,.T.);
#47321=EDGE_CURVE('',#38014,#38015,#31117,.T.);
#47322=EDGE_CURVE('',#38015,#38012,#20583,.T.);
#47323=EDGE_CURVE('',#37508,#37997,#31118,.T.);
#47324=EDGE_CURVE('',#37996,#37509,#31119,.T.);
#47325=EDGE_CURVE('',#38014,#37064,#470,.T.);
#47326=EDGE_CURVE('',#37063,#38015,#471,.T.);
#47327=EDGE_CURVE('',#38006,#38009,#472,.T.);
#47328=EDGE_CURVE('',#38008,#38007,#473,.T.);
#47329=EDGE_CURVE('',#38002,#38005,#474,.T.);
#47330=EDGE_CURVE('',#38004,#38003,#475,.T.);
#47331=EDGE_CURVE('',#38016,#38017,#31120,.T.);
#47332=EDGE_CURVE('',#38017,#38018,#20584,.T.);
#47333=EDGE_CURVE('',#38019,#38018,#31121,.T.);
#47334=EDGE_CURVE('',#38020,#38019,#31122,.T.);
#47335=EDGE_CURVE('',#38021,#38020,#31123,.T.);
#47336=EDGE_CURVE('',#38021,#38016,#20585,.T.);
#47337=EDGE_CURVE('',#38019,#38022,#20586,.T.);
#47338=EDGE_CURVE('',#38022,#38023,#31124,.T.);
#47339=EDGE_CURVE('',#38023,#38020,#20587,.T.);
#47340=EDGE_CURVE('',#38024,#38025,#31125,.T.);
#47341=EDGE_CURVE('',#38025,#38026,#20588,.T.);
#47342=EDGE_CURVE('',#38026,#38027,#31126,.T.);
#47343=EDGE_CURVE('',#38027,#38024,#20589,.T.);
#47344=EDGE_CURVE('',#38028,#38029,#31127,.T.);
#47345=EDGE_CURVE('',#38029,#38030,#20590,.T.);
#47346=EDGE_CURVE('',#38031,#38030,#31128,.T.);
#47347=EDGE_CURVE('',#38032,#38031,#31129,.T.);
#47348=EDGE_CURVE('',#38033,#38032,#31130,.T.);
#47349=EDGE_CURVE('',#38033,#38028,#20591,.T.);
#47350=EDGE_CURVE('',#38031,#38034,#20592,.T.);
#47351=EDGE_CURVE('',#38034,#38035,#31131,.T.);
#47352=EDGE_CURVE('',#38035,#38032,#20593,.T.);
#47353=EDGE_CURVE('',#37514,#38017,#31132,.T.);
#47354=EDGE_CURVE('',#38016,#37515,#31133,.T.);
#47355=EDGE_CURVE('',#38034,#37058,#476,.T.);
#47356=EDGE_CURVE('',#37057,#38035,#477,.T.);
#47357=EDGE_CURVE('',#38026,#38029,#478,.T.);
#47358=EDGE_CURVE('',#38028,#38027,#479,.T.);
#47359=EDGE_CURVE('',#38022,#38025,#480,.T.);
#47360=EDGE_CURVE('',#38024,#38023,#481,.T.);
#47361=EDGE_CURVE('',#38036,#38037,#31134,.T.);
#47362=EDGE_CURVE('',#38037,#38038,#20594,.T.);
#47363=EDGE_CURVE('',#38039,#38038,#31135,.T.);
#47364=EDGE_CURVE('',#38040,#38039,#31136,.T.);
#47365=EDGE_CURVE('',#38041,#38040,#31137,.T.);
#47366=EDGE_CURVE('',#38041,#38036,#20595,.T.);
#47367=EDGE_CURVE('',#38039,#38042,#20596,.T.);
#47368=EDGE_CURVE('',#38042,#38043,#31138,.T.);
#47369=EDGE_CURVE('',#38043,#38040,#20597,.T.);
#47370=EDGE_CURVE('',#38044,#38045,#31139,.T.);
#47371=EDGE_CURVE('',#38045,#38046,#20598,.T.);
#47372=EDGE_CURVE('',#38046,#38047,#31140,.T.);
#47373=EDGE_CURVE('',#38047,#38044,#20599,.T.);
#47374=EDGE_CURVE('',#38048,#38049,#31141,.T.);
#47375=EDGE_CURVE('',#38049,#38050,#20600,.T.);
#47376=EDGE_CURVE('',#38051,#38050,#31142,.T.);
#47377=EDGE_CURVE('',#38052,#38051,#31143,.T.);
#47378=EDGE_CURVE('',#38053,#38052,#31144,.T.);
#47379=EDGE_CURVE('',#38053,#38048,#20601,.T.);
#47380=EDGE_CURVE('',#38051,#38054,#20602,.T.);
#47381=EDGE_CURVE('',#38054,#38055,#31145,.T.);
#47382=EDGE_CURVE('',#38055,#38052,#20603,.T.);
#47383=EDGE_CURVE('',#37520,#38037,#31146,.T.);
#47384=EDGE_CURVE('',#38036,#37521,#31147,.T.);
#47385=EDGE_CURVE('',#38054,#37052,#482,.T.);
#47386=EDGE_CURVE('',#37051,#38055,#483,.T.);
#47387=EDGE_CURVE('',#38046,#38049,#484,.T.);
#47388=EDGE_CURVE('',#38048,#38047,#485,.T.);
#47389=EDGE_CURVE('',#38042,#38045,#486,.T.);
#47390=EDGE_CURVE('',#38044,#38043,#487,.T.);
#47391=EDGE_CURVE('',#38056,#38057,#31148,.T.);
#47392=EDGE_CURVE('',#38057,#38058,#20604,.T.);
#47393=EDGE_CURVE('',#38059,#38058,#31149,.T.);
#47394=EDGE_CURVE('',#38060,#38059,#31150,.T.);
#47395=EDGE_CURVE('',#38061,#38060,#31151,.T.);
#47396=EDGE_CURVE('',#38061,#38056,#20605,.T.);
#47397=EDGE_CURVE('',#38059,#38062,#20606,.T.);
#47398=EDGE_CURVE('',#38062,#38063,#31152,.T.);
#47399=EDGE_CURVE('',#38063,#38060,#20607,.T.);
#47400=EDGE_CURVE('',#38064,#38065,#31153,.T.);
#47401=EDGE_CURVE('',#38065,#38066,#20608,.T.);
#47402=EDGE_CURVE('',#38066,#38067,#31154,.T.);
#47403=EDGE_CURVE('',#38067,#38064,#20609,.T.);
#47404=EDGE_CURVE('',#38068,#38069,#31155,.T.);
#47405=EDGE_CURVE('',#38069,#38070,#20610,.T.);
#47406=EDGE_CURVE('',#38071,#38070,#31156,.T.);
#47407=EDGE_CURVE('',#38072,#38071,#31157,.T.);
#47408=EDGE_CURVE('',#38073,#38072,#31158,.T.);
#47409=EDGE_CURVE('',#38073,#38068,#20611,.T.);
#47410=EDGE_CURVE('',#38071,#38074,#20612,.T.);
#47411=EDGE_CURVE('',#38074,#38075,#31159,.T.);
#47412=EDGE_CURVE('',#38075,#38072,#20613,.T.);
#47413=EDGE_CURVE('',#37526,#38057,#31160,.T.);
#47414=EDGE_CURVE('',#38056,#37527,#31161,.T.);
#47415=EDGE_CURVE('',#38074,#37046,#488,.T.);
#47416=EDGE_CURVE('',#37045,#38075,#489,.T.);
#47417=EDGE_CURVE('',#38066,#38069,#490,.T.);
#47418=EDGE_CURVE('',#38068,#38067,#491,.T.);
#47419=EDGE_CURVE('',#38062,#38065,#492,.T.);
#47420=EDGE_CURVE('',#38064,#38063,#493,.T.);
#47421=EDGE_CURVE('',#38076,#38077,#31162,.T.);
#47422=EDGE_CURVE('',#38077,#38078,#20614,.T.);
#47423=EDGE_CURVE('',#38079,#38078,#31163,.T.);
#47424=EDGE_CURVE('',#38080,#38079,#31164,.T.);
#47425=EDGE_CURVE('',#38081,#38080,#31165,.T.);
#47426=EDGE_CURVE('',#38081,#38076,#20615,.T.);
#47427=EDGE_CURVE('',#38079,#38082,#20616,.T.);
#47428=EDGE_CURVE('',#38082,#38083,#31166,.T.);
#47429=EDGE_CURVE('',#38083,#38080,#20617,.T.);
#47430=EDGE_CURVE('',#38084,#38085,#31167,.T.);
#47431=EDGE_CURVE('',#38085,#38086,#20618,.T.);
#47432=EDGE_CURVE('',#38086,#38087,#31168,.T.);
#47433=EDGE_CURVE('',#38087,#38084,#20619,.T.);
#47434=EDGE_CURVE('',#38088,#38089,#31169,.T.);
#47435=EDGE_CURVE('',#38089,#38090,#20620,.T.);
#47436=EDGE_CURVE('',#38091,#38090,#31170,.T.);
#47437=EDGE_CURVE('',#38092,#38091,#31171,.T.);
#47438=EDGE_CURVE('',#38093,#38092,#31172,.T.);
#47439=EDGE_CURVE('',#38093,#38088,#20621,.T.);
#47440=EDGE_CURVE('',#38091,#38094,#20622,.T.);
#47441=EDGE_CURVE('',#38094,#38095,#31173,.T.);
#47442=EDGE_CURVE('',#38095,#38092,#20623,.T.);
#47443=EDGE_CURVE('',#37532,#38077,#31174,.T.);
#47444=EDGE_CURVE('',#38076,#37533,#31175,.T.);
#47445=EDGE_CURVE('',#38094,#37040,#494,.T.);
#47446=EDGE_CURVE('',#37039,#38095,#495,.T.);
#47447=EDGE_CURVE('',#38086,#38089,#496,.T.);
#47448=EDGE_CURVE('',#38088,#38087,#497,.T.);
#47449=EDGE_CURVE('',#38082,#38085,#498,.T.);
#47450=EDGE_CURVE('',#38084,#38083,#499,.T.);
#47451=EDGE_CURVE('',#38096,#38097,#31176,.T.);
#47452=EDGE_CURVE('',#38097,#38098,#20624,.T.);
#47453=EDGE_CURVE('',#38099,#38098,#31177,.T.);
#47454=EDGE_CURVE('',#38100,#38099,#31178,.T.);
#47455=EDGE_CURVE('',#38101,#38100,#31179,.T.);
#47456=EDGE_CURVE('',#38101,#38096,#20625,.T.);
#47457=EDGE_CURVE('',#38099,#38102,#20626,.T.);
#47458=EDGE_CURVE('',#38102,#38103,#31180,.T.);
#47459=EDGE_CURVE('',#38103,#38100,#20627,.T.);
#47460=EDGE_CURVE('',#38104,#38105,#31181,.T.);
#47461=EDGE_CURVE('',#38105,#38106,#20628,.T.);
#47462=EDGE_CURVE('',#38106,#38107,#31182,.T.);
#47463=EDGE_CURVE('',#38107,#38104,#20629,.T.);
#47464=EDGE_CURVE('',#38108,#38109,#31183,.T.);
#47465=EDGE_CURVE('',#38109,#38110,#20630,.T.);
#47466=EDGE_CURVE('',#38111,#38110,#31184,.T.);
#47467=EDGE_CURVE('',#38112,#38111,#31185,.T.);
#47468=EDGE_CURVE('',#38113,#38112,#31186,.T.);
#47469=EDGE_CURVE('',#38113,#38108,#20631,.T.);
#47470=EDGE_CURVE('',#38111,#38114,#20632,.T.);
#47471=EDGE_CURVE('',#38114,#38115,#31187,.T.);
#47472=EDGE_CURVE('',#38115,#38112,#20633,.T.);
#47473=EDGE_CURVE('',#37538,#38097,#31188,.T.);
#47474=EDGE_CURVE('',#38096,#37539,#31189,.T.);
#47475=EDGE_CURVE('',#38114,#37034,#500,.T.);
#47476=EDGE_CURVE('',#37033,#38115,#501,.T.);
#47477=EDGE_CURVE('',#38106,#38109,#502,.T.);
#47478=EDGE_CURVE('',#38108,#38107,#503,.T.);
#47479=EDGE_CURVE('',#38102,#38105,#504,.T.);
#47480=EDGE_CURVE('',#38104,#38103,#505,.T.);
#47481=EDGE_CURVE('',#38116,#38117,#31190,.T.);
#47482=EDGE_CURVE('',#38117,#38118,#20634,.T.);
#47483=EDGE_CURVE('',#38119,#38118,#31191,.T.);
#47484=EDGE_CURVE('',#38120,#38119,#31192,.T.);
#47485=EDGE_CURVE('',#38121,#38120,#31193,.T.);
#47486=EDGE_CURVE('',#38121,#38116,#20635,.T.);
#47487=EDGE_CURVE('',#38119,#38122,#20636,.T.);
#47488=EDGE_CURVE('',#38122,#38123,#31194,.T.);
#47489=EDGE_CURVE('',#38123,#38120,#20637,.T.);
#47490=EDGE_CURVE('',#38124,#38125,#31195,.T.);
#47491=EDGE_CURVE('',#38125,#38126,#20638,.T.);
#47492=EDGE_CURVE('',#38126,#38127,#31196,.T.);
#47493=EDGE_CURVE('',#38127,#38124,#20639,.T.);
#47494=EDGE_CURVE('',#38128,#38129,#31197,.T.);
#47495=EDGE_CURVE('',#38129,#38130,#20640,.T.);
#47496=EDGE_CURVE('',#38131,#38130,#31198,.T.);
#47497=EDGE_CURVE('',#38132,#38131,#31199,.T.);
#47498=EDGE_CURVE('',#38133,#38132,#31200,.T.);
#47499=EDGE_CURVE('',#38133,#38128,#20641,.T.);
#47500=EDGE_CURVE('',#38131,#38134,#20642,.T.);
#47501=EDGE_CURVE('',#38134,#38135,#31201,.T.);
#47502=EDGE_CURVE('',#38135,#38132,#20643,.T.);
#47503=EDGE_CURVE('',#37544,#38117,#31202,.T.);
#47504=EDGE_CURVE('',#38116,#37545,#31203,.T.);
#47505=EDGE_CURVE('',#38134,#37028,#506,.T.);
#47506=EDGE_CURVE('',#37027,#38135,#507,.T.);
#47507=EDGE_CURVE('',#38126,#38129,#508,.T.);
#47508=EDGE_CURVE('',#38128,#38127,#509,.T.);
#47509=EDGE_CURVE('',#38122,#38125,#510,.T.);
#47510=EDGE_CURVE('',#38124,#38123,#511,.T.);
#47511=EDGE_CURVE('',#38136,#38137,#31204,.T.);
#47512=EDGE_CURVE('',#38137,#38138,#20644,.T.);
#47513=EDGE_CURVE('',#38139,#38138,#31205,.T.);
#47514=EDGE_CURVE('',#38140,#38139,#31206,.T.);
#47515=EDGE_CURVE('',#38141,#38140,#31207,.T.);
#47516=EDGE_CURVE('',#38141,#38136,#20645,.T.);
#47517=EDGE_CURVE('',#38139,#38142,#20646,.T.);
#47518=EDGE_CURVE('',#38142,#38143,#31208,.T.);
#47519=EDGE_CURVE('',#38143,#38140,#20647,.T.);
#47520=EDGE_CURVE('',#38144,#38145,#31209,.T.);
#47521=EDGE_CURVE('',#38145,#38146,#20648,.T.);
#47522=EDGE_CURVE('',#38146,#38147,#31210,.T.);
#47523=EDGE_CURVE('',#38147,#38144,#20649,.T.);
#47524=EDGE_CURVE('',#38148,#38149,#31211,.T.);
#47525=EDGE_CURVE('',#38149,#38150,#20650,.T.);
#47526=EDGE_CURVE('',#38151,#38150,#31212,.T.);
#47527=EDGE_CURVE('',#38152,#38151,#31213,.T.);
#47528=EDGE_CURVE('',#38153,#38152,#31214,.T.);
#47529=EDGE_CURVE('',#38153,#38148,#20651,.T.);
#47530=EDGE_CURVE('',#38151,#38154,#20652,.T.);
#47531=EDGE_CURVE('',#38154,#38155,#31215,.T.);
#47532=EDGE_CURVE('',#38155,#38152,#20653,.T.);
#47533=EDGE_CURVE('',#37550,#38137,#31216,.T.);
#47534=EDGE_CURVE('',#38136,#37551,#31217,.T.);
#47535=EDGE_CURVE('',#38154,#37022,#512,.T.);
#47536=EDGE_CURVE('',#37021,#38155,#513,.T.);
#47537=EDGE_CURVE('',#38146,#38149,#514,.T.);
#47538=EDGE_CURVE('',#38148,#38147,#515,.T.);
#47539=EDGE_CURVE('',#38142,#38145,#516,.T.);
#47540=EDGE_CURVE('',#38144,#38143,#517,.T.);
#47541=EDGE_CURVE('',#38156,#38157,#31218,.T.);
#47542=EDGE_CURVE('',#38157,#38158,#20654,.T.);
#47543=EDGE_CURVE('',#38159,#38158,#31219,.T.);
#47544=EDGE_CURVE('',#38160,#38159,#31220,.T.);
#47545=EDGE_CURVE('',#38161,#38160,#31221,.T.);
#47546=EDGE_CURVE('',#38161,#38156,#20655,.T.);
#47547=EDGE_CURVE('',#38159,#38162,#20656,.T.);
#47548=EDGE_CURVE('',#38162,#38163,#31222,.T.);
#47549=EDGE_CURVE('',#38163,#38160,#20657,.T.);
#47550=EDGE_CURVE('',#38164,#38165,#31223,.T.);
#47551=EDGE_CURVE('',#38165,#38166,#20658,.T.);
#47552=EDGE_CURVE('',#38166,#38167,#31224,.T.);
#47553=EDGE_CURVE('',#38167,#38164,#20659,.T.);
#47554=EDGE_CURVE('',#38168,#38169,#31225,.T.);
#47555=EDGE_CURVE('',#38169,#38170,#20660,.T.);
#47556=EDGE_CURVE('',#38171,#38170,#31226,.T.);
#47557=EDGE_CURVE('',#38172,#38171,#31227,.T.);
#47558=EDGE_CURVE('',#38173,#38172,#31228,.T.);
#47559=EDGE_CURVE('',#38173,#38168,#20661,.T.);
#47560=EDGE_CURVE('',#38171,#38174,#20662,.T.);
#47561=EDGE_CURVE('',#38174,#38175,#31229,.T.);
#47562=EDGE_CURVE('',#38175,#38172,#20663,.T.);
#47563=EDGE_CURVE('',#37197,#38157,#31230,.T.);
#47564=EDGE_CURVE('',#38156,#37198,#31231,.T.);
#47565=EDGE_CURVE('',#38174,#37018,#518,.T.);
#47566=EDGE_CURVE('',#37017,#38175,#519,.T.);
#47567=EDGE_CURVE('',#38166,#38169,#520,.T.);
#47568=EDGE_CURVE('',#38168,#38167,#521,.T.);
#47569=EDGE_CURVE('',#38162,#38165,#522,.T.);
#47570=EDGE_CURVE('',#38164,#38163,#523,.T.);
#47571=EDGE_CURVE('',#38176,#38177,#31232,.T.);
#47572=EDGE_CURVE('',#38177,#38178,#20664,.T.);
#47573=EDGE_CURVE('',#38179,#38178,#31233,.T.);
#47574=EDGE_CURVE('',#38180,#38179,#31234,.T.);
#47575=EDGE_CURVE('',#38181,#38180,#31235,.T.);
#47576=EDGE_CURVE('',#38181,#38176,#20665,.T.);
#47577=EDGE_CURVE('',#38179,#38182,#20666,.T.);
#47578=EDGE_CURVE('',#38182,#38183,#31236,.T.);
#47579=EDGE_CURVE('',#38183,#38180,#20667,.T.);
#47580=EDGE_CURVE('',#38184,#38185,#31237,.T.);
#47581=EDGE_CURVE('',#38185,#38186,#20668,.T.);
#47582=EDGE_CURVE('',#38186,#38187,#31238,.T.);
#47583=EDGE_CURVE('',#38187,#38184,#20669,.T.);
#47584=EDGE_CURVE('',#38188,#38189,#31239,.T.);
#47585=EDGE_CURVE('',#38189,#38190,#20670,.T.);
#47586=EDGE_CURVE('',#38191,#38190,#31240,.T.);
#47587=EDGE_CURVE('',#38192,#38191,#31241,.T.);
#47588=EDGE_CURVE('',#38193,#38192,#31242,.T.);
#47589=EDGE_CURVE('',#38193,#38188,#20671,.T.);
#47590=EDGE_CURVE('',#38191,#38194,#20672,.T.);
#47591=EDGE_CURVE('',#38194,#38195,#31243,.T.);
#47592=EDGE_CURVE('',#38195,#38192,#20673,.T.);
#47593=EDGE_CURVE('',#37203,#38177,#31244,.T.);
#47594=EDGE_CURVE('',#38176,#37204,#31245,.T.);
#47595=EDGE_CURVE('',#38194,#37012,#524,.T.);
#47596=EDGE_CURVE('',#37011,#38195,#525,.T.);
#47597=EDGE_CURVE('',#38186,#38189,#526,.T.);
#47598=EDGE_CURVE('',#38188,#38187,#527,.T.);
#47599=EDGE_CURVE('',#38182,#38185,#528,.T.);
#47600=EDGE_CURVE('',#38184,#38183,#529,.T.);
#47601=EDGE_CURVE('',#38196,#38197,#31246,.T.);
#47602=EDGE_CURVE('',#38197,#38198,#20674,.T.);
#47603=EDGE_CURVE('',#38199,#38198,#31247,.T.);
#47604=EDGE_CURVE('',#38200,#38199,#31248,.T.);
#47605=EDGE_CURVE('',#38201,#38200,#31249,.T.);
#47606=EDGE_CURVE('',#38201,#38196,#20675,.T.);
#47607=EDGE_CURVE('',#38199,#38202,#20676,.T.);
#47608=EDGE_CURVE('',#38202,#38203,#31250,.T.);
#47609=EDGE_CURVE('',#38203,#38200,#20677,.T.);
#47610=EDGE_CURVE('',#38204,#38205,#31251,.T.);
#47611=EDGE_CURVE('',#38205,#38206,#20678,.T.);
#47612=EDGE_CURVE('',#38206,#38207,#31252,.T.);
#47613=EDGE_CURVE('',#38207,#38204,#20679,.T.);
#47614=EDGE_CURVE('',#38208,#38209,#31253,.T.);
#47615=EDGE_CURVE('',#38209,#38210,#20680,.T.);
#47616=EDGE_CURVE('',#38211,#38210,#31254,.T.);
#47617=EDGE_CURVE('',#38212,#38211,#31255,.T.);
#47618=EDGE_CURVE('',#38213,#38212,#31256,.T.);
#47619=EDGE_CURVE('',#38213,#38208,#20681,.T.);
#47620=EDGE_CURVE('',#38211,#38214,#20682,.T.);
#47621=EDGE_CURVE('',#38214,#38215,#31257,.T.);
#47622=EDGE_CURVE('',#38215,#38212,#20683,.T.);
#47623=EDGE_CURVE('',#37209,#38197,#31258,.T.);
#47624=EDGE_CURVE('',#38196,#37210,#31259,.T.);
#47625=EDGE_CURVE('',#38214,#37006,#530,.T.);
#47626=EDGE_CURVE('',#37005,#38215,#531,.T.);
#47627=EDGE_CURVE('',#38206,#38209,#532,.T.);
#47628=EDGE_CURVE('',#38208,#38207,#533,.T.);
#47629=EDGE_CURVE('',#38202,#38205,#534,.T.);
#47630=EDGE_CURVE('',#38204,#38203,#535,.T.);
#47631=EDGE_CURVE('',#38216,#38217,#31260,.T.);
#47632=EDGE_CURVE('',#38217,#38218,#20684,.T.);
#47633=EDGE_CURVE('',#38219,#38218,#31261,.T.);
#47634=EDGE_CURVE('',#38220,#38219,#31262,.T.);
#47635=EDGE_CURVE('',#38221,#38220,#31263,.T.);
#47636=EDGE_CURVE('',#38221,#38216,#20685,.T.);
#47637=EDGE_CURVE('',#38219,#38222,#20686,.T.);
#47638=EDGE_CURVE('',#38222,#38223,#31264,.T.);
#47639=EDGE_CURVE('',#38223,#38220,#20687,.T.);
#47640=EDGE_CURVE('',#38224,#38225,#31265,.T.);
#47641=EDGE_CURVE('',#38225,#38226,#20688,.T.);
#47642=EDGE_CURVE('',#38226,#38227,#31266,.T.);
#47643=EDGE_CURVE('',#38227,#38224,#20689,.T.);
#47644=EDGE_CURVE('',#38228,#38229,#31267,.T.);
#47645=EDGE_CURVE('',#38229,#38230,#20690,.T.);
#47646=EDGE_CURVE('',#38231,#38230,#31268,.T.);
#47647=EDGE_CURVE('',#38232,#38231,#31269,.T.);
#47648=EDGE_CURVE('',#38233,#38232,#31270,.T.);
#47649=EDGE_CURVE('',#38233,#38228,#20691,.T.);
#47650=EDGE_CURVE('',#38231,#38234,#20692,.T.);
#47651=EDGE_CURVE('',#38234,#38235,#31271,.T.);
#47652=EDGE_CURVE('',#38235,#38232,#20693,.T.);
#47653=EDGE_CURVE('',#37215,#38217,#31272,.T.);
#47654=EDGE_CURVE('',#38216,#37216,#31273,.T.);
#47655=EDGE_CURVE('',#38234,#37000,#536,.T.);
#47656=EDGE_CURVE('',#36999,#38235,#537,.T.);
#47657=EDGE_CURVE('',#38226,#38229,#538,.T.);
#47658=EDGE_CURVE('',#38228,#38227,#539,.T.);
#47659=EDGE_CURVE('',#38222,#38225,#540,.T.);
#47660=EDGE_CURVE('',#38224,#38223,#541,.T.);
#47661=EDGE_CURVE('',#38236,#38237,#31274,.T.);
#47662=EDGE_CURVE('',#38237,#38238,#20694,.T.);
#47663=EDGE_CURVE('',#38239,#38238,#31275,.T.);
#47664=EDGE_CURVE('',#38240,#38239,#31276,.T.);
#47665=EDGE_CURVE('',#38241,#38240,#31277,.T.);
#47666=EDGE_CURVE('',#38241,#38236,#20695,.T.);
#47667=EDGE_CURVE('',#38239,#38242,#20696,.T.);
#47668=EDGE_CURVE('',#38242,#38243,#31278,.T.);
#47669=EDGE_CURVE('',#38243,#38240,#20697,.T.);
#47670=EDGE_CURVE('',#38244,#38245,#31279,.T.);
#47671=EDGE_CURVE('',#38245,#38246,#20698,.T.);
#47672=EDGE_CURVE('',#38246,#38247,#31280,.T.);
#47673=EDGE_CURVE('',#38247,#38244,#20699,.T.);
#47674=EDGE_CURVE('',#38248,#38249,#31281,.T.);
#47675=EDGE_CURVE('',#38249,#38250,#20700,.T.);
#47676=EDGE_CURVE('',#38251,#38250,#31282,.T.);
#47677=EDGE_CURVE('',#38252,#38251,#31283,.T.);
#47678=EDGE_CURVE('',#38253,#38252,#31284,.T.);
#47679=EDGE_CURVE('',#38253,#38248,#20701,.T.);
#47680=EDGE_CURVE('',#38251,#38254,#20702,.T.);
#47681=EDGE_CURVE('',#38254,#38255,#31285,.T.);
#47682=EDGE_CURVE('',#38255,#38252,#20703,.T.);
#47683=EDGE_CURVE('',#37221,#38237,#31286,.T.);
#47684=EDGE_CURVE('',#38236,#37222,#31287,.T.);
#47685=EDGE_CURVE('',#38254,#36994,#542,.T.);
#47686=EDGE_CURVE('',#36993,#38255,#543,.T.);
#47687=EDGE_CURVE('',#38246,#38249,#544,.T.);
#47688=EDGE_CURVE('',#38248,#38247,#545,.T.);
#47689=EDGE_CURVE('',#38242,#38245,#546,.T.);
#47690=EDGE_CURVE('',#38244,#38243,#547,.T.);
#47691=EDGE_CURVE('',#38256,#38257,#31288,.T.);
#47692=EDGE_CURVE('',#38257,#38258,#20704,.T.);
#47693=EDGE_CURVE('',#38259,#38258,#31289,.T.);
#47694=EDGE_CURVE('',#38260,#38259,#31290,.T.);
#47695=EDGE_CURVE('',#38261,#38260,#31291,.T.);
#47696=EDGE_CURVE('',#38261,#38256,#20705,.T.);
#47697=EDGE_CURVE('',#38259,#38262,#20706,.T.);
#47698=EDGE_CURVE('',#38262,#38263,#31292,.T.);
#47699=EDGE_CURVE('',#38263,#38260,#20707,.T.);
#47700=EDGE_CURVE('',#38264,#38265,#31293,.T.);
#47701=EDGE_CURVE('',#38265,#38266,#20708,.T.);
#47702=EDGE_CURVE('',#38266,#38267,#31294,.T.);
#47703=EDGE_CURVE('',#38267,#38264,#20709,.T.);
#47704=EDGE_CURVE('',#38268,#38269,#31295,.T.);
#47705=EDGE_CURVE('',#38269,#38270,#20710,.T.);
#47706=EDGE_CURVE('',#38271,#38270,#31296,.T.);
#47707=EDGE_CURVE('',#38272,#38271,#31297,.T.);
#47708=EDGE_CURVE('',#38273,#38272,#31298,.T.);
#47709=EDGE_CURVE('',#38273,#38268,#20711,.T.);
#47710=EDGE_CURVE('',#38271,#38274,#20712,.T.);
#47711=EDGE_CURVE('',#38274,#38275,#31299,.T.);
#47712=EDGE_CURVE('',#38275,#38272,#20713,.T.);
#47713=EDGE_CURVE('',#37227,#38257,#31300,.T.);
#47714=EDGE_CURVE('',#38256,#37228,#31301,.T.);
#47715=EDGE_CURVE('',#38274,#36988,#548,.T.);
#47716=EDGE_CURVE('',#36987,#38275,#549,.T.);
#47717=EDGE_CURVE('',#38266,#38269,#550,.T.);
#47718=EDGE_CURVE('',#38268,#38267,#551,.T.);
#47719=EDGE_CURVE('',#38262,#38265,#552,.T.);
#47720=EDGE_CURVE('',#38264,#38263,#553,.T.);
#47721=EDGE_CURVE('',#38276,#38277,#31302,.T.);
#47722=EDGE_CURVE('',#38277,#38278,#20714,.T.);
#47723=EDGE_CURVE('',#38279,#38278,#31303,.T.);
#47724=EDGE_CURVE('',#38280,#38279,#31304,.T.);
#47725=EDGE_CURVE('',#38281,#38280,#31305,.T.);
#47726=EDGE_CURVE('',#38281,#38276,#20715,.T.);
#47727=EDGE_CURVE('',#38279,#38282,#20716,.T.);
#47728=EDGE_CURVE('',#38282,#38283,#31306,.T.);
#47729=EDGE_CURVE('',#38283,#38280,#20717,.T.);
#47730=EDGE_CURVE('',#38284,#38285,#31307,.T.);
#47731=EDGE_CURVE('',#38285,#38286,#20718,.T.);
#47732=EDGE_CURVE('',#38286,#38287,#31308,.T.);
#47733=EDGE_CURVE('',#38287,#38284,#20719,.T.);
#47734=EDGE_CURVE('',#38288,#38289,#31309,.T.);
#47735=EDGE_CURVE('',#38289,#38290,#20720,.T.);
#47736=EDGE_CURVE('',#38291,#38290,#31310,.T.);
#47737=EDGE_CURVE('',#38292,#38291,#31311,.T.);
#47738=EDGE_CURVE('',#38293,#38292,#31312,.T.);
#47739=EDGE_CURVE('',#38293,#38288,#20721,.T.);
#47740=EDGE_CURVE('',#38291,#38294,#20722,.T.);
#47741=EDGE_CURVE('',#38294,#38295,#31313,.T.);
#47742=EDGE_CURVE('',#38295,#38292,#20723,.T.);
#47743=EDGE_CURVE('',#37233,#38277,#31314,.T.);
#47744=EDGE_CURVE('',#38276,#37234,#31315,.T.);
#47745=EDGE_CURVE('',#38294,#36982,#554,.T.);
#47746=EDGE_CURVE('',#36981,#38295,#555,.T.);
#47747=EDGE_CURVE('',#38286,#38289,#556,.T.);
#47748=EDGE_CURVE('',#38288,#38287,#557,.T.);
#47749=EDGE_CURVE('',#38282,#38285,#558,.T.);
#47750=EDGE_CURVE('',#38284,#38283,#559,.T.);
#47751=EDGE_CURVE('',#38296,#38297,#31316,.T.);
#47752=EDGE_CURVE('',#38297,#38298,#20724,.T.);
#47753=EDGE_CURVE('',#38299,#38298,#31317,.T.);
#47754=EDGE_CURVE('',#38300,#38299,#31318,.T.);
#47755=EDGE_CURVE('',#38301,#38300,#31319,.T.);
#47756=EDGE_CURVE('',#38301,#38296,#20725,.T.);
#47757=EDGE_CURVE('',#38299,#38302,#20726,.T.);
#47758=EDGE_CURVE('',#38302,#38303,#31320,.T.);
#47759=EDGE_CURVE('',#38303,#38300,#20727,.T.);
#47760=EDGE_CURVE('',#38304,#38305,#31321,.T.);
#47761=EDGE_CURVE('',#38305,#38306,#20728,.T.);
#47762=EDGE_CURVE('',#38306,#38307,#31322,.T.);
#47763=EDGE_CURVE('',#38307,#38304,#20729,.T.);
#47764=EDGE_CURVE('',#38308,#38309,#31323,.T.);
#47765=EDGE_CURVE('',#38309,#38310,#20730,.T.);
#47766=EDGE_CURVE('',#38311,#38310,#31324,.T.);
#47767=EDGE_CURVE('',#38312,#38311,#31325,.T.);
#47768=EDGE_CURVE('',#38313,#38312,#31326,.T.);
#47769=EDGE_CURVE('',#38313,#38308,#20731,.T.);
#47770=EDGE_CURVE('',#38311,#38314,#20732,.T.);
#47771=EDGE_CURVE('',#38314,#38315,#31327,.T.);
#47772=EDGE_CURVE('',#38315,#38312,#20733,.T.);
#47773=EDGE_CURVE('',#37239,#38297,#31328,.T.);
#47774=EDGE_CURVE('',#38296,#37240,#31329,.T.);
#47775=EDGE_CURVE('',#38314,#36976,#560,.T.);
#47776=EDGE_CURVE('',#36975,#38315,#561,.T.);
#47777=EDGE_CURVE('',#38306,#38309,#562,.T.);
#47778=EDGE_CURVE('',#38308,#38307,#563,.T.);
#47779=EDGE_CURVE('',#38302,#38305,#564,.T.);
#47780=EDGE_CURVE('',#38304,#38303,#565,.T.);
#47781=EDGE_CURVE('',#38316,#38317,#31330,.T.);
#47782=EDGE_CURVE('',#38317,#38318,#20734,.T.);
#47783=EDGE_CURVE('',#38319,#38318,#31331,.T.);
#47784=EDGE_CURVE('',#38320,#38319,#31332,.T.);
#47785=EDGE_CURVE('',#38321,#38320,#31333,.T.);
#47786=EDGE_CURVE('',#38321,#38316,#20735,.T.);
#47787=EDGE_CURVE('',#38319,#38322,#20736,.T.);
#47788=EDGE_CURVE('',#38322,#38323,#31334,.T.);
#47789=EDGE_CURVE('',#38323,#38320,#20737,.T.);
#47790=EDGE_CURVE('',#38324,#38325,#31335,.T.);
#47791=EDGE_CURVE('',#38325,#38326,#20738,.T.);
#47792=EDGE_CURVE('',#38326,#38327,#31336,.T.);
#47793=EDGE_CURVE('',#38327,#38324,#20739,.T.);
#47794=EDGE_CURVE('',#38328,#38329,#31337,.T.);
#47795=EDGE_CURVE('',#38329,#38330,#20740,.T.);
#47796=EDGE_CURVE('',#38331,#38330,#31338,.T.);
#47797=EDGE_CURVE('',#38332,#38331,#31339,.T.);
#47798=EDGE_CURVE('',#38333,#38332,#31340,.T.);
#47799=EDGE_CURVE('',#38333,#38328,#20741,.T.);
#47800=EDGE_CURVE('',#38331,#38334,#20742,.T.);
#47801=EDGE_CURVE('',#38334,#38335,#31341,.T.);
#47802=EDGE_CURVE('',#38335,#38332,#20743,.T.);
#47803=EDGE_CURVE('',#37245,#38317,#31342,.T.);
#47804=EDGE_CURVE('',#38316,#37246,#31343,.T.);
#47805=EDGE_CURVE('',#38334,#36970,#566,.T.);
#47806=EDGE_CURVE('',#36969,#38335,#567,.T.);
#47807=EDGE_CURVE('',#38326,#38329,#568,.T.);
#47808=EDGE_CURVE('',#38328,#38327,#569,.T.);
#47809=EDGE_CURVE('',#38322,#38325,#570,.T.);
#47810=EDGE_CURVE('',#38324,#38323,#571,.T.);
#47811=EDGE_CURVE('',#38336,#38337,#31344,.T.);
#47812=EDGE_CURVE('',#38337,#38338,#20744,.T.);
#47813=EDGE_CURVE('',#38339,#38338,#31345,.T.);
#47814=EDGE_CURVE('',#38340,#38339,#31346,.T.);
#47815=EDGE_CURVE('',#38341,#38340,#31347,.T.);
#47816=EDGE_CURVE('',#38341,#38336,#20745,.T.);
#47817=EDGE_CURVE('',#38339,#38342,#20746,.T.);
#47818=EDGE_CURVE('',#38342,#38343,#31348,.T.);
#47819=EDGE_CURVE('',#38343,#38340,#20747,.T.);
#47820=EDGE_CURVE('',#38344,#38345,#31349,.T.);
#47821=EDGE_CURVE('',#38345,#38346,#20748,.T.);
#47822=EDGE_CURVE('',#38346,#38347,#31350,.T.);
#47823=EDGE_CURVE('',#38347,#38344,#20749,.T.);
#47824=EDGE_CURVE('',#38348,#38349,#31351,.T.);
#47825=EDGE_CURVE('',#38349,#38350,#20750,.T.);
#47826=EDGE_CURVE('',#38351,#38350,#31352,.T.);
#47827=EDGE_CURVE('',#38352,#38351,#31353,.T.);
#47828=EDGE_CURVE('',#38353,#38352,#31354,.T.);
#47829=EDGE_CURVE('',#38353,#38348,#20751,.T.);
#47830=EDGE_CURVE('',#38351,#38354,#20752,.T.);
#47831=EDGE_CURVE('',#38354,#38355,#31355,.T.);
#47832=EDGE_CURVE('',#38355,#38352,#20753,.T.);
#47833=EDGE_CURVE('',#37251,#38337,#31356,.T.);
#47834=EDGE_CURVE('',#38336,#37252,#31357,.T.);
#47835=EDGE_CURVE('',#38354,#36964,#572,.T.);
#47836=EDGE_CURVE('',#36963,#38355,#573,.T.);
#47837=EDGE_CURVE('',#38346,#38349,#574,.T.);
#47838=EDGE_CURVE('',#38348,#38347,#575,.T.);
#47839=EDGE_CURVE('',#38342,#38345,#576,.T.);
#47840=EDGE_CURVE('',#38344,#38343,#577,.T.);
#47841=EDGE_CURVE('',#38356,#38357,#31358,.T.);
#47842=EDGE_CURVE('',#38357,#38358,#20754,.T.);
#47843=EDGE_CURVE('',#38359,#38358,#31359,.T.);
#47844=EDGE_CURVE('',#38360,#38359,#31360,.T.);
#47845=EDGE_CURVE('',#38361,#38360,#31361,.T.);
#47846=EDGE_CURVE('',#38361,#38356,#20755,.T.);
#47847=EDGE_CURVE('',#38359,#38362,#20756,.T.);
#47848=EDGE_CURVE('',#38362,#38363,#31362,.T.);
#47849=EDGE_CURVE('',#38363,#38360,#20757,.T.);
#47850=EDGE_CURVE('',#38364,#38365,#31363,.T.);
#47851=EDGE_CURVE('',#38365,#38366,#20758,.T.);
#47852=EDGE_CURVE('',#38366,#38367,#31364,.T.);
#47853=EDGE_CURVE('',#38367,#38364,#20759,.T.);
#47854=EDGE_CURVE('',#38368,#38369,#31365,.T.);
#47855=EDGE_CURVE('',#38369,#38370,#20760,.T.);
#47856=EDGE_CURVE('',#38371,#38370,#31366,.T.);
#47857=EDGE_CURVE('',#38372,#38371,#31367,.T.);
#47858=EDGE_CURVE('',#38373,#38372,#31368,.T.);
#47859=EDGE_CURVE('',#38373,#38368,#20761,.T.);
#47860=EDGE_CURVE('',#38371,#38374,#20762,.T.);
#47861=EDGE_CURVE('',#38374,#38375,#31369,.T.);
#47862=EDGE_CURVE('',#38375,#38372,#20763,.T.);
#47863=EDGE_CURVE('',#37257,#38357,#31370,.T.);
#47864=EDGE_CURVE('',#38356,#37258,#31371,.T.);
#47865=EDGE_CURVE('',#38374,#36958,#578,.T.);
#47866=EDGE_CURVE('',#36957,#38375,#579,.T.);
#47867=EDGE_CURVE('',#38366,#38369,#580,.T.);
#47868=EDGE_CURVE('',#38368,#38367,#581,.T.);
#47869=EDGE_CURVE('',#38362,#38365,#582,.T.);
#47870=EDGE_CURVE('',#38364,#38363,#583,.T.);
#47871=EDGE_CURVE('',#38376,#38377,#31372,.T.);
#47872=EDGE_CURVE('',#38377,#38378,#20764,.T.);
#47873=EDGE_CURVE('',#38379,#38378,#31373,.T.);
#47874=EDGE_CURVE('',#38380,#38379,#31374,.T.);
#47875=EDGE_CURVE('',#38381,#38380,#31375,.T.);
#47876=EDGE_CURVE('',#38381,#38376,#20765,.T.);
#47877=EDGE_CURVE('',#38379,#38382,#20766,.T.);
#47878=EDGE_CURVE('',#38382,#38383,#31376,.T.);
#47879=EDGE_CURVE('',#38383,#38380,#20767,.T.);
#47880=EDGE_CURVE('',#38384,#38385,#31377,.T.);
#47881=EDGE_CURVE('',#38385,#38386,#20768,.T.);
#47882=EDGE_CURVE('',#38386,#38387,#31378,.T.);
#47883=EDGE_CURVE('',#38387,#38384,#20769,.T.);
#47884=EDGE_CURVE('',#38388,#38389,#31379,.T.);
#47885=EDGE_CURVE('',#38389,#38390,#20770,.T.);
#47886=EDGE_CURVE('',#38391,#38390,#31380,.T.);
#47887=EDGE_CURVE('',#38392,#38391,#31381,.T.);
#47888=EDGE_CURVE('',#38393,#38392,#31382,.T.);
#47889=EDGE_CURVE('',#38393,#38388,#20771,.T.);
#47890=EDGE_CURVE('',#38391,#38394,#20772,.T.);
#47891=EDGE_CURVE('',#38394,#38395,#31383,.T.);
#47892=EDGE_CURVE('',#38395,#38392,#20773,.T.);
#47893=EDGE_CURVE('',#37263,#38377,#31384,.T.);
#47894=EDGE_CURVE('',#38376,#37264,#31385,.T.);
#47895=EDGE_CURVE('',#38394,#36952,#584,.T.);
#47896=EDGE_CURVE('',#36951,#38395,#585,.T.);
#47897=EDGE_CURVE('',#38386,#38389,#586,.T.);
#47898=EDGE_CURVE('',#38388,#38387,#587,.T.);
#47899=EDGE_CURVE('',#38382,#38385,#588,.T.);
#47900=EDGE_CURVE('',#38384,#38383,#589,.T.);
#47901=EDGE_CURVE('',#38396,#38397,#31386,.T.);
#47902=EDGE_CURVE('',#38397,#38398,#20774,.T.);
#47903=EDGE_CURVE('',#38399,#38398,#31387,.T.);
#47904=EDGE_CURVE('',#38400,#38399,#31388,.T.);
#47905=EDGE_CURVE('',#38401,#38400,#31389,.T.);
#47906=EDGE_CURVE('',#38401,#38396,#20775,.T.);
#47907=EDGE_CURVE('',#38399,#38402,#20776,.T.);
#47908=EDGE_CURVE('',#38402,#38403,#31390,.T.);
#47909=EDGE_CURVE('',#38403,#38400,#20777,.T.);
#47910=EDGE_CURVE('',#38404,#38405,#31391,.T.);
#47911=EDGE_CURVE('',#38405,#38406,#20778,.T.);
#47912=EDGE_CURVE('',#38406,#38407,#31392,.T.);
#47913=EDGE_CURVE('',#38407,#38404,#20779,.T.);
#47914=EDGE_CURVE('',#38408,#38409,#31393,.T.);
#47915=EDGE_CURVE('',#38409,#38410,#20780,.T.);
#47916=EDGE_CURVE('',#38411,#38410,#31394,.T.);
#47917=EDGE_CURVE('',#38412,#38411,#31395,.T.);
#47918=EDGE_CURVE('',#38413,#38412,#31396,.T.);
#47919=EDGE_CURVE('',#38413,#38408,#20781,.T.);
#47920=EDGE_CURVE('',#38411,#38414,#20782,.T.);
#47921=EDGE_CURVE('',#38414,#38415,#31397,.T.);
#47922=EDGE_CURVE('',#38415,#38412,#20783,.T.);
#47923=EDGE_CURVE('',#37269,#38397,#31398,.T.);
#47924=EDGE_CURVE('',#38396,#37270,#31399,.T.);
#47925=EDGE_CURVE('',#38414,#36946,#590,.T.);
#47926=EDGE_CURVE('',#36945,#38415,#591,.T.);
#47927=EDGE_CURVE('',#38406,#38409,#592,.T.);
#47928=EDGE_CURVE('',#38408,#38407,#593,.T.);
#47929=EDGE_CURVE('',#38402,#38405,#594,.T.);
#47930=EDGE_CURVE('',#38404,#38403,#595,.T.);
#47931=EDGE_CURVE('',#38416,#38417,#31400,.T.);
#47932=EDGE_CURVE('',#38417,#38418,#20784,.T.);
#47933=EDGE_CURVE('',#38419,#38418,#31401,.T.);
#47934=EDGE_CURVE('',#38420,#38419,#31402,.T.);
#47935=EDGE_CURVE('',#38421,#38420,#31403,.T.);
#47936=EDGE_CURVE('',#38421,#38416,#20785,.T.);
#47937=EDGE_CURVE('',#38419,#38422,#20786,.T.);
#47938=EDGE_CURVE('',#38422,#38423,#31404,.T.);
#47939=EDGE_CURVE('',#38423,#38420,#20787,.T.);
#47940=EDGE_CURVE('',#38424,#38425,#31405,.T.);
#47941=EDGE_CURVE('',#38425,#38426,#20788,.T.);
#47942=EDGE_CURVE('',#38426,#38427,#31406,.T.);
#47943=EDGE_CURVE('',#38427,#38424,#20789,.T.);
#47944=EDGE_CURVE('',#38428,#38429,#31407,.T.);
#47945=EDGE_CURVE('',#38429,#38430,#20790,.T.);
#47946=EDGE_CURVE('',#38431,#38430,#31408,.T.);
#47947=EDGE_CURVE('',#38432,#38431,#31409,.T.);
#47948=EDGE_CURVE('',#38433,#38432,#31410,.T.);
#47949=EDGE_CURVE('',#38433,#38428,#20791,.T.);
#47950=EDGE_CURVE('',#38431,#38434,#20792,.T.);
#47951=EDGE_CURVE('',#38434,#38435,#31411,.T.);
#47952=EDGE_CURVE('',#38435,#38432,#20793,.T.);
#47953=EDGE_CURVE('',#37275,#38417,#31412,.T.);
#47954=EDGE_CURVE('',#38416,#37276,#31413,.T.);
#47955=EDGE_CURVE('',#38434,#36940,#596,.T.);
#47956=EDGE_CURVE('',#36939,#38435,#597,.T.);
#47957=EDGE_CURVE('',#38426,#38429,#598,.T.);
#47958=EDGE_CURVE('',#38428,#38427,#599,.T.);
#47959=EDGE_CURVE('',#38422,#38425,#600,.T.);
#47960=EDGE_CURVE('',#38424,#38423,#601,.T.);
#47961=EDGE_CURVE('',#38436,#38437,#31414,.T.);
#47962=EDGE_CURVE('',#38437,#38438,#20794,.T.);
#47963=EDGE_CURVE('',#38439,#38438,#31415,.T.);
#47964=EDGE_CURVE('',#38440,#38439,#31416,.T.);
#47965=EDGE_CURVE('',#38441,#38440,#31417,.T.);
#47966=EDGE_CURVE('',#38441,#38436,#20795,.T.);
#47967=EDGE_CURVE('',#38439,#38442,#20796,.T.);
#47968=EDGE_CURVE('',#38442,#38443,#31418,.T.);
#47969=EDGE_CURVE('',#38443,#38440,#20797,.T.);
#47970=EDGE_CURVE('',#38444,#38445,#31419,.T.);
#47971=EDGE_CURVE('',#38445,#38446,#20798,.T.);
#47972=EDGE_CURVE('',#38446,#38447,#31420,.T.);
#47973=EDGE_CURVE('',#38447,#38444,#20799,.T.);
#47974=EDGE_CURVE('',#38448,#38449,#31421,.T.);
#47975=EDGE_CURVE('',#38449,#38450,#20800,.T.);
#47976=EDGE_CURVE('',#38451,#38450,#31422,.T.);
#47977=EDGE_CURVE('',#38452,#38451,#31423,.T.);
#47978=EDGE_CURVE('',#38453,#38452,#31424,.T.);
#47979=EDGE_CURVE('',#38453,#38448,#20801,.T.);
#47980=EDGE_CURVE('',#38451,#38454,#20802,.T.);
#47981=EDGE_CURVE('',#38454,#38455,#31425,.T.);
#47982=EDGE_CURVE('',#38455,#38452,#20803,.T.);
#47983=EDGE_CURVE('',#37281,#38437,#31426,.T.);
#47984=EDGE_CURVE('',#38436,#37282,#31427,.T.);
#47985=EDGE_CURVE('',#38454,#36934,#602,.T.);
#47986=EDGE_CURVE('',#36933,#38455,#603,.T.);
#47987=EDGE_CURVE('',#38446,#38449,#604,.T.);
#47988=EDGE_CURVE('',#38448,#38447,#605,.T.);
#47989=EDGE_CURVE('',#38442,#38445,#606,.T.);
#47990=EDGE_CURVE('',#38444,#38443,#607,.T.);
#47991=EDGE_CURVE('',#38456,#38457,#31428,.T.);
#47992=EDGE_CURVE('',#38457,#38458,#20804,.T.);
#47993=EDGE_CURVE('',#38459,#38458,#31429,.T.);
#47994=EDGE_CURVE('',#38460,#38459,#31430,.T.);
#47995=EDGE_CURVE('',#38461,#38460,#31431,.T.);
#47996=EDGE_CURVE('',#38461,#38456,#20805,.T.);
#47997=EDGE_CURVE('',#38459,#38462,#20806,.T.);
#47998=EDGE_CURVE('',#38462,#38463,#31432,.T.);
#47999=EDGE_CURVE('',#38463,#38460,#20807,.T.);
#48000=EDGE_CURVE('',#38464,#38465,#31433,.T.);
#48001=EDGE_CURVE('',#38465,#38466,#20808,.T.);
#48002=EDGE_CURVE('',#38466,#38467,#31434,.T.);
#48003=EDGE_CURVE('',#38467,#38464,#20809,.T.);
#48004=EDGE_CURVE('',#38468,#38469,#31435,.T.);
#48005=EDGE_CURVE('',#38469,#38470,#20810,.T.);
#48006=EDGE_CURVE('',#38471,#38470,#31436,.T.);
#48007=EDGE_CURVE('',#38472,#38471,#31437,.T.);
#48008=EDGE_CURVE('',#38473,#38472,#31438,.T.);
#48009=EDGE_CURVE('',#38473,#38468,#20811,.T.);
#48010=EDGE_CURVE('',#38471,#38474,#20812,.T.);
#48011=EDGE_CURVE('',#38474,#38475,#31439,.T.);
#48012=EDGE_CURVE('',#38475,#38472,#20813,.T.);
#48013=EDGE_CURVE('',#37287,#38457,#31440,.T.);
#48014=EDGE_CURVE('',#38456,#37288,#31441,.T.);
#48015=EDGE_CURVE('',#38474,#36928,#608,.T.);
#48016=EDGE_CURVE('',#36927,#38475,#609,.T.);
#48017=EDGE_CURVE('',#38466,#38469,#610,.T.);
#48018=EDGE_CURVE('',#38468,#38467,#611,.T.);
#48019=EDGE_CURVE('',#38462,#38465,#612,.T.);
#48020=EDGE_CURVE('',#38464,#38463,#613,.T.);
#48021=EDGE_CURVE('',#38476,#38477,#31442,.T.);
#48022=EDGE_CURVE('',#38477,#38478,#20814,.T.);
#48023=EDGE_CURVE('',#38479,#38478,#31443,.T.);
#48024=EDGE_CURVE('',#38480,#38479,#31444,.T.);
#48025=EDGE_CURVE('',#38481,#38480,#31445,.T.);
#48026=EDGE_CURVE('',#38481,#38476,#20815,.T.);
#48027=EDGE_CURVE('',#38479,#38482,#20816,.T.);
#48028=EDGE_CURVE('',#38482,#38483,#31446,.T.);
#48029=EDGE_CURVE('',#38483,#38480,#20817,.T.);
#48030=EDGE_CURVE('',#38484,#38485,#31447,.T.);
#48031=EDGE_CURVE('',#38485,#38486,#20818,.T.);
#48032=EDGE_CURVE('',#38486,#38487,#31448,.T.);
#48033=EDGE_CURVE('',#38487,#38484,#20819,.T.);
#48034=EDGE_CURVE('',#38488,#38489,#31449,.T.);
#48035=EDGE_CURVE('',#38489,#38490,#20820,.T.);
#48036=EDGE_CURVE('',#38491,#38490,#31450,.T.);
#48037=EDGE_CURVE('',#38492,#38491,#31451,.T.);
#48038=EDGE_CURVE('',#38493,#38492,#31452,.T.);
#48039=EDGE_CURVE('',#38493,#38488,#20821,.T.);
#48040=EDGE_CURVE('',#38491,#38494,#20822,.T.);
#48041=EDGE_CURVE('',#38494,#38495,#31453,.T.);
#48042=EDGE_CURVE('',#38495,#38492,#20823,.T.);
#48043=EDGE_CURVE('',#37293,#38477,#31454,.T.);
#48044=EDGE_CURVE('',#38476,#37294,#31455,.T.);
#48045=EDGE_CURVE('',#38494,#36922,#614,.T.);
#48046=EDGE_CURVE('',#36921,#38495,#615,.T.);
#48047=EDGE_CURVE('',#38486,#38489,#616,.T.);
#48048=EDGE_CURVE('',#38488,#38487,#617,.T.);
#48049=EDGE_CURVE('',#38482,#38485,#618,.T.);
#48050=EDGE_CURVE('',#38484,#38483,#619,.T.);
#48051=EDGE_CURVE('',#38496,#38497,#31456,.T.);
#48052=EDGE_CURVE('',#38497,#38498,#20824,.T.);
#48053=EDGE_CURVE('',#38499,#38498,#31457,.T.);
#48054=EDGE_CURVE('',#38500,#38499,#31458,.T.);
#48055=EDGE_CURVE('',#38501,#38500,#31459,.T.);
#48056=EDGE_CURVE('',#38501,#38496,#20825,.T.);
#48057=EDGE_CURVE('',#38499,#38502,#20826,.T.);
#48058=EDGE_CURVE('',#38502,#38503,#31460,.T.);
#48059=EDGE_CURVE('',#38503,#38500,#20827,.T.);
#48060=EDGE_CURVE('',#38504,#38505,#31461,.T.);
#48061=EDGE_CURVE('',#38505,#38506,#20828,.T.);
#48062=EDGE_CURVE('',#38506,#38507,#31462,.T.);
#48063=EDGE_CURVE('',#38507,#38504,#20829,.T.);
#48064=EDGE_CURVE('',#38508,#38509,#31463,.T.);
#48065=EDGE_CURVE('',#38509,#38510,#20830,.T.);
#48066=EDGE_CURVE('',#38511,#38510,#31464,.T.);
#48067=EDGE_CURVE('',#38512,#38511,#31465,.T.);
#48068=EDGE_CURVE('',#38513,#38512,#31466,.T.);
#48069=EDGE_CURVE('',#38513,#38508,#20831,.T.);
#48070=EDGE_CURVE('',#38511,#38514,#20832,.T.);
#48071=EDGE_CURVE('',#38514,#38515,#31467,.T.);
#48072=EDGE_CURVE('',#38515,#38512,#20833,.T.);
#48073=EDGE_CURVE('',#37299,#38497,#31468,.T.);
#48074=EDGE_CURVE('',#38496,#37300,#31469,.T.);
#48075=EDGE_CURVE('',#38514,#36916,#620,.T.);
#48076=EDGE_CURVE('',#36915,#38515,#621,.T.);
#48077=EDGE_CURVE('',#38506,#38509,#622,.T.);
#48078=EDGE_CURVE('',#38508,#38507,#623,.T.);
#48079=EDGE_CURVE('',#38502,#38505,#624,.T.);
#48080=EDGE_CURVE('',#38504,#38503,#625,.T.);
#48081=EDGE_CURVE('',#38516,#38517,#31470,.T.);
#48082=EDGE_CURVE('',#38517,#38518,#20834,.T.);
#48083=EDGE_CURVE('',#38519,#38518,#31471,.T.);
#48084=EDGE_CURVE('',#38520,#38519,#31472,.T.);
#48085=EDGE_CURVE('',#38521,#38520,#31473,.T.);
#48086=EDGE_CURVE('',#38521,#38516,#20835,.T.);
#48087=EDGE_CURVE('',#38519,#38522,#20836,.T.);
#48088=EDGE_CURVE('',#38522,#38523,#31474,.T.);
#48089=EDGE_CURVE('',#38523,#38520,#20837,.T.);
#48090=EDGE_CURVE('',#38524,#38525,#31475,.T.);
#48091=EDGE_CURVE('',#38525,#38526,#20838,.T.);
#48092=EDGE_CURVE('',#38526,#38527,#31476,.T.);
#48093=EDGE_CURVE('',#38527,#38524,#20839,.T.);
#48094=EDGE_CURVE('',#38528,#38529,#31477,.T.);
#48095=EDGE_CURVE('',#38529,#38530,#20840,.T.);
#48096=EDGE_CURVE('',#38531,#38530,#31478,.T.);
#48097=EDGE_CURVE('',#38532,#38531,#31479,.T.);
#48098=EDGE_CURVE('',#38533,#38532,#31480,.T.);
#48099=EDGE_CURVE('',#38533,#38528,#20841,.T.);
#48100=EDGE_CURVE('',#38531,#38534,#20842,.T.);
#48101=EDGE_CURVE('',#38534,#38535,#31481,.T.);
#48102=EDGE_CURVE('',#38535,#38532,#20843,.T.);
#48103=EDGE_CURVE('',#37305,#38517,#31482,.T.);
#48104=EDGE_CURVE('',#38516,#37306,#31483,.T.);
#48105=EDGE_CURVE('',#38534,#36910,#626,.T.);
#48106=EDGE_CURVE('',#36909,#38535,#627,.T.);
#48107=EDGE_CURVE('',#38526,#38529,#628,.T.);
#48108=EDGE_CURVE('',#38528,#38527,#629,.T.);
#48109=EDGE_CURVE('',#38522,#38525,#630,.T.);
#48110=EDGE_CURVE('',#38524,#38523,#631,.T.);
#48111=EDGE_CURVE('',#38536,#38537,#31484,.T.);
#48112=EDGE_CURVE('',#38537,#38538,#20844,.T.);
#48113=EDGE_CURVE('',#38539,#38538,#31485,.T.);
#48114=EDGE_CURVE('',#38540,#38539,#31486,.T.);
#48115=EDGE_CURVE('',#38541,#38540,#31487,.T.);
#48116=EDGE_CURVE('',#38541,#38536,#20845,.T.);
#48117=EDGE_CURVE('',#38539,#38542,#20846,.T.);
#48118=EDGE_CURVE('',#38542,#38543,#31488,.T.);
#48119=EDGE_CURVE('',#38543,#38540,#20847,.T.);
#48120=EDGE_CURVE('',#38544,#38545,#31489,.T.);
#48121=EDGE_CURVE('',#38545,#38546,#20848,.T.);
#48122=EDGE_CURVE('',#38546,#38547,#31490,.T.);
#48123=EDGE_CURVE('',#38547,#38544,#20849,.T.);
#48124=EDGE_CURVE('',#38548,#38549,#31491,.T.);
#48125=EDGE_CURVE('',#38549,#38550,#20850,.T.);
#48126=EDGE_CURVE('',#38551,#38550,#31492,.T.);
#48127=EDGE_CURVE('',#38552,#38551,#31493,.T.);
#48128=EDGE_CURVE('',#38553,#38552,#31494,.T.);
#48129=EDGE_CURVE('',#38553,#38548,#20851,.T.);
#48130=EDGE_CURVE('',#38551,#38554,#20852,.T.);
#48131=EDGE_CURVE('',#38554,#38555,#31495,.T.);
#48132=EDGE_CURVE('',#38555,#38552,#20853,.T.);
#48133=EDGE_CURVE('',#37311,#38537,#31496,.T.);
#48134=EDGE_CURVE('',#38536,#37312,#31497,.T.);
#48135=EDGE_CURVE('',#38554,#36904,#632,.T.);
#48136=EDGE_CURVE('',#36903,#38555,#633,.T.);
#48137=EDGE_CURVE('',#38546,#38549,#634,.T.);
#48138=EDGE_CURVE('',#38548,#38547,#635,.T.);
#48139=EDGE_CURVE('',#38542,#38545,#636,.T.);
#48140=EDGE_CURVE('',#38544,#38543,#637,.T.);
#48141=EDGE_CURVE('',#38556,#38557,#31498,.T.);
#48142=EDGE_CURVE('',#38557,#38558,#20854,.T.);
#48143=EDGE_CURVE('',#38559,#38558,#31499,.T.);
#48144=EDGE_CURVE('',#38560,#38559,#31500,.T.);
#48145=EDGE_CURVE('',#38561,#38560,#31501,.T.);
#48146=EDGE_CURVE('',#38561,#38556,#20855,.T.);
#48147=EDGE_CURVE('',#38559,#38562,#20856,.T.);
#48148=EDGE_CURVE('',#38562,#38563,#31502,.T.);
#48149=EDGE_CURVE('',#38563,#38560,#20857,.T.);
#48150=EDGE_CURVE('',#38564,#38565,#31503,.T.);
#48151=EDGE_CURVE('',#38565,#38566,#20858,.T.);
#48152=EDGE_CURVE('',#38566,#38567,#31504,.T.);
#48153=EDGE_CURVE('',#38567,#38564,#20859,.T.);
#48154=EDGE_CURVE('',#38568,#38569,#31505,.T.);
#48155=EDGE_CURVE('',#38569,#38570,#20860,.T.);
#48156=EDGE_CURVE('',#38571,#38570,#31506,.T.);
#48157=EDGE_CURVE('',#38572,#38571,#31507,.T.);
#48158=EDGE_CURVE('',#38573,#38572,#31508,.T.);
#48159=EDGE_CURVE('',#38573,#38568,#20861,.T.);
#48160=EDGE_CURVE('',#38571,#38574,#20862,.T.);
#48161=EDGE_CURVE('',#38574,#38575,#31509,.T.);
#48162=EDGE_CURVE('',#38575,#38572,#20863,.T.);
#48163=EDGE_CURVE('',#37317,#38557,#31510,.T.);
#48164=EDGE_CURVE('',#38556,#37318,#31511,.T.);
#48165=EDGE_CURVE('',#38574,#36898,#638,.T.);
#48166=EDGE_CURVE('',#36897,#38575,#639,.T.);
#48167=EDGE_CURVE('',#38566,#38569,#640,.T.);
#48168=EDGE_CURVE('',#38568,#38567,#641,.T.);
#48169=EDGE_CURVE('',#38562,#38565,#642,.T.);
#48170=EDGE_CURVE('',#38564,#38563,#643,.T.);
#48171=EDGE_CURVE('',#38576,#38577,#31512,.T.);
#48172=EDGE_CURVE('',#38577,#38578,#20864,.T.);
#48173=EDGE_CURVE('',#38579,#38578,#31513,.T.);
#48174=EDGE_CURVE('',#38580,#38579,#31514,.T.);
#48175=EDGE_CURVE('',#38581,#38580,#31515,.T.);
#48176=EDGE_CURVE('',#38581,#38576,#20865,.T.);
#48177=EDGE_CURVE('',#38579,#38582,#20866,.T.);
#48178=EDGE_CURVE('',#38582,#38583,#31516,.T.);
#48179=EDGE_CURVE('',#38583,#38580,#20867,.T.);
#48180=EDGE_CURVE('',#38584,#38585,#31517,.T.);
#48181=EDGE_CURVE('',#38585,#38586,#20868,.T.);
#48182=EDGE_CURVE('',#38586,#38587,#31518,.T.);
#48183=EDGE_CURVE('',#38587,#38584,#20869,.T.);
#48184=EDGE_CURVE('',#38588,#38589,#31519,.T.);
#48185=EDGE_CURVE('',#38589,#38590,#20870,.T.);
#48186=EDGE_CURVE('',#38591,#38590,#31520,.T.);
#48187=EDGE_CURVE('',#38592,#38591,#31521,.T.);
#48188=EDGE_CURVE('',#38593,#38592,#31522,.T.);
#48189=EDGE_CURVE('',#38593,#38588,#20871,.T.);
#48190=EDGE_CURVE('',#38591,#38594,#20872,.T.);
#48191=EDGE_CURVE('',#38594,#38595,#31523,.T.);
#48192=EDGE_CURVE('',#38595,#38592,#20873,.T.);
#48193=EDGE_CURVE('',#37323,#38577,#31524,.T.);
#48194=EDGE_CURVE('',#38576,#37324,#31525,.T.);
#48195=EDGE_CURVE('',#38594,#36892,#644,.T.);
#48196=EDGE_CURVE('',#36891,#38595,#645,.T.);
#48197=EDGE_CURVE('',#38586,#38589,#646,.T.);
#48198=EDGE_CURVE('',#38588,#38587,#647,.T.);
#48199=EDGE_CURVE('',#38582,#38585,#648,.T.);
#48200=EDGE_CURVE('',#38584,#38583,#649,.T.);
#48201=EDGE_CURVE('',#38596,#38597,#31526,.T.);
#48202=EDGE_CURVE('',#38597,#38598,#20874,.T.);
#48203=EDGE_CURVE('',#38599,#38598,#31527,.T.);
#48204=EDGE_CURVE('',#38600,#38599,#31528,.T.);
#48205=EDGE_CURVE('',#38601,#38600,#31529,.T.);
#48206=EDGE_CURVE('',#38601,#38596,#20875,.T.);
#48207=EDGE_CURVE('',#38599,#38602,#20876,.T.);
#48208=EDGE_CURVE('',#38602,#38603,#31530,.T.);
#48209=EDGE_CURVE('',#38603,#38600,#20877,.T.);
#48210=EDGE_CURVE('',#38604,#38605,#31531,.T.);
#48211=EDGE_CURVE('',#38605,#38606,#20878,.T.);
#48212=EDGE_CURVE('',#38606,#38607,#31532,.T.);
#48213=EDGE_CURVE('',#38607,#38604,#20879,.T.);
#48214=EDGE_CURVE('',#38608,#38609,#31533,.T.);
#48215=EDGE_CURVE('',#38609,#38610,#20880,.T.);
#48216=EDGE_CURVE('',#38611,#38610,#31534,.T.);
#48217=EDGE_CURVE('',#38612,#38611,#31535,.T.);
#48218=EDGE_CURVE('',#38613,#38612,#31536,.T.);
#48219=EDGE_CURVE('',#38613,#38608,#20881,.T.);
#48220=EDGE_CURVE('',#38611,#38614,#20882,.T.);
#48221=EDGE_CURVE('',#38614,#38615,#31537,.T.);
#48222=EDGE_CURVE('',#38615,#38612,#20883,.T.);
#48223=EDGE_CURVE('',#37329,#38597,#31538,.T.);
#48224=EDGE_CURVE('',#38596,#37330,#31539,.T.);
#48225=EDGE_CURVE('',#38614,#36886,#650,.T.);
#48226=EDGE_CURVE('',#36885,#38615,#651,.T.);
#48227=EDGE_CURVE('',#38606,#38609,#652,.T.);
#48228=EDGE_CURVE('',#38608,#38607,#653,.T.);
#48229=EDGE_CURVE('',#38602,#38605,#654,.T.);
#48230=EDGE_CURVE('',#38604,#38603,#655,.T.);
#48231=EDGE_CURVE('',#38616,#38617,#31540,.T.);
#48232=EDGE_CURVE('',#38617,#38618,#20884,.T.);
#48233=EDGE_CURVE('',#38619,#38618,#31541,.T.);
#48234=EDGE_CURVE('',#38620,#38619,#31542,.T.);
#48235=EDGE_CURVE('',#38621,#38620,#31543,.T.);
#48236=EDGE_CURVE('',#38621,#38616,#20885,.T.);
#48237=EDGE_CURVE('',#38619,#38622,#20886,.T.);
#48238=EDGE_CURVE('',#38622,#38623,#31544,.T.);
#48239=EDGE_CURVE('',#38623,#38620,#20887,.T.);
#48240=EDGE_CURVE('',#38624,#38625,#31545,.T.);
#48241=EDGE_CURVE('',#38625,#38626,#20888,.T.);
#48242=EDGE_CURVE('',#38626,#38627,#31546,.T.);
#48243=EDGE_CURVE('',#38627,#38624,#20889,.T.);
#48244=EDGE_CURVE('',#38628,#38629,#31547,.T.);
#48245=EDGE_CURVE('',#38629,#38630,#20890,.T.);
#48246=EDGE_CURVE('',#38631,#38630,#31548,.T.);
#48247=EDGE_CURVE('',#38632,#38631,#31549,.T.);
#48248=EDGE_CURVE('',#38633,#38632,#31550,.T.);
#48249=EDGE_CURVE('',#38633,#38628,#20891,.T.);
#48250=EDGE_CURVE('',#38631,#38634,#20892,.T.);
#48251=EDGE_CURVE('',#38634,#38635,#31551,.T.);
#48252=EDGE_CURVE('',#38635,#38632,#20893,.T.);
#48253=EDGE_CURVE('',#37335,#38617,#31552,.T.);
#48254=EDGE_CURVE('',#38616,#37336,#31553,.T.);
#48255=EDGE_CURVE('',#38634,#36880,#656,.T.);
#48256=EDGE_CURVE('',#36879,#38635,#657,.T.);
#48257=EDGE_CURVE('',#38626,#38629,#658,.T.);
#48258=EDGE_CURVE('',#38628,#38627,#659,.T.);
#48259=EDGE_CURVE('',#38622,#38625,#660,.T.);
#48260=EDGE_CURVE('',#38624,#38623,#661,.T.);
#48261=EDGE_CURVE('',#38636,#38637,#31554,.T.);
#48262=EDGE_CURVE('',#38637,#38638,#20894,.T.);
#48263=EDGE_CURVE('',#38639,#38638,#31555,.T.);
#48264=EDGE_CURVE('',#38640,#38639,#31556,.T.);
#48265=EDGE_CURVE('',#38641,#38640,#31557,.T.);
#48266=EDGE_CURVE('',#38641,#38636,#20895,.T.);
#48267=EDGE_CURVE('',#38639,#38642,#20896,.T.);
#48268=EDGE_CURVE('',#38642,#38643,#31558,.T.);
#48269=EDGE_CURVE('',#38643,#38640,#20897,.T.);
#48270=EDGE_CURVE('',#38644,#38645,#31559,.T.);
#48271=EDGE_CURVE('',#38645,#38646,#20898,.T.);
#48272=EDGE_CURVE('',#38646,#38647,#31560,.T.);
#48273=EDGE_CURVE('',#38647,#38644,#20899,.T.);
#48274=EDGE_CURVE('',#38648,#38649,#31561,.T.);
#48275=EDGE_CURVE('',#38649,#38650,#20900,.T.);
#48276=EDGE_CURVE('',#38651,#38650,#31562,.T.);
#48277=EDGE_CURVE('',#38652,#38651,#31563,.T.);
#48278=EDGE_CURVE('',#38653,#38652,#31564,.T.);
#48279=EDGE_CURVE('',#38653,#38648,#20901,.T.);
#48280=EDGE_CURVE('',#38651,#38654,#20902,.T.);
#48281=EDGE_CURVE('',#38654,#38655,#31565,.T.);
#48282=EDGE_CURVE('',#38655,#38652,#20903,.T.);
#48283=EDGE_CURVE('',#37341,#38637,#31566,.T.);
#48284=EDGE_CURVE('',#38636,#37342,#31567,.T.);
#48285=EDGE_CURVE('',#38654,#36874,#662,.T.);
#48286=EDGE_CURVE('',#36873,#38655,#663,.T.);
#48287=EDGE_CURVE('',#38646,#38649,#664,.T.);
#48288=EDGE_CURVE('',#38648,#38647,#665,.T.);
#48289=EDGE_CURVE('',#38642,#38645,#666,.T.);
#48290=EDGE_CURVE('',#38644,#38643,#667,.T.);
#48291=EDGE_CURVE('',#38656,#38657,#31568,.T.);
#48292=EDGE_CURVE('',#38657,#38658,#20904,.T.);
#48293=EDGE_CURVE('',#38659,#38658,#31569,.T.);
#48294=EDGE_CURVE('',#38660,#38659,#31570,.T.);
#48295=EDGE_CURVE('',#38661,#38660,#31571,.T.);
#48296=EDGE_CURVE('',#38661,#38656,#20905,.T.);
#48297=EDGE_CURVE('',#38659,#38662,#20906,.T.);
#48298=EDGE_CURVE('',#38662,#38663,#31572,.T.);
#48299=EDGE_CURVE('',#38663,#38660,#20907,.T.);
#48300=EDGE_CURVE('',#38664,#38665,#31573,.T.);
#48301=EDGE_CURVE('',#38665,#38666,#20908,.T.);
#48302=EDGE_CURVE('',#38666,#38667,#31574,.T.);
#48303=EDGE_CURVE('',#38667,#38664,#20909,.T.);
#48304=EDGE_CURVE('',#38668,#38669,#31575,.T.);
#48305=EDGE_CURVE('',#38669,#38670,#20910,.T.);
#48306=EDGE_CURVE('',#38671,#38670,#31576,.T.);
#48307=EDGE_CURVE('',#38672,#38671,#31577,.T.);
#48308=EDGE_CURVE('',#38673,#38672,#31578,.T.);
#48309=EDGE_CURVE('',#38673,#38668,#20911,.T.);
#48310=EDGE_CURVE('',#38671,#38674,#20912,.T.);
#48311=EDGE_CURVE('',#38674,#38675,#31579,.T.);
#48312=EDGE_CURVE('',#38675,#38672,#20913,.T.);
#48313=EDGE_CURVE('',#37347,#38657,#31580,.T.);
#48314=EDGE_CURVE('',#38656,#37348,#31581,.T.);
#48315=EDGE_CURVE('',#38674,#36868,#668,.T.);
#48316=EDGE_CURVE('',#36867,#38675,#669,.T.);
#48317=EDGE_CURVE('',#38666,#38669,#670,.T.);
#48318=EDGE_CURVE('',#38668,#38667,#671,.T.);
#48319=EDGE_CURVE('',#38662,#38665,#672,.T.);
#48320=EDGE_CURVE('',#38664,#38663,#673,.T.);
#48321=EDGE_CURVE('',#38676,#38677,#31582,.T.);
#48322=EDGE_CURVE('',#38677,#38678,#20914,.T.);
#48323=EDGE_CURVE('',#38679,#38678,#31583,.T.);
#48324=EDGE_CURVE('',#38680,#38679,#31584,.T.);
#48325=EDGE_CURVE('',#38681,#38680,#31585,.T.);
#48326=EDGE_CURVE('',#38681,#38676,#20915,.T.);
#48327=EDGE_CURVE('',#38679,#38682,#20916,.T.);
#48328=EDGE_CURVE('',#38682,#38683,#31586,.T.);
#48329=EDGE_CURVE('',#38683,#38680,#20917,.T.);
#48330=EDGE_CURVE('',#38684,#38685,#31587,.T.);
#48331=EDGE_CURVE('',#38685,#38686,#20918,.T.);
#48332=EDGE_CURVE('',#38686,#38687,#31588,.T.);
#48333=EDGE_CURVE('',#38687,#38684,#20919,.T.);
#48334=EDGE_CURVE('',#38688,#38689,#31589,.T.);
#48335=EDGE_CURVE('',#38689,#38690,#20920,.T.);
#48336=EDGE_CURVE('',#38691,#38690,#31590,.T.);
#48337=EDGE_CURVE('',#38692,#38691,#31591,.T.);
#48338=EDGE_CURVE('',#38693,#38692,#31592,.T.);
#48339=EDGE_CURVE('',#38693,#38688,#20921,.T.);
#48340=EDGE_CURVE('',#38691,#38694,#20922,.T.);
#48341=EDGE_CURVE('',#38694,#38695,#31593,.T.);
#48342=EDGE_CURVE('',#38695,#38692,#20923,.T.);
#48343=EDGE_CURVE('',#37353,#38677,#31594,.T.);
#48344=EDGE_CURVE('',#38676,#37354,#31595,.T.);
#48345=EDGE_CURVE('',#38694,#36862,#674,.T.);
#48346=EDGE_CURVE('',#36861,#38695,#675,.T.);
#48347=EDGE_CURVE('',#38686,#38689,#676,.T.);
#48348=EDGE_CURVE('',#38688,#38687,#677,.T.);
#48349=EDGE_CURVE('',#38682,#38685,#678,.T.);
#48350=EDGE_CURVE('',#38684,#38683,#679,.T.);
#48351=EDGE_CURVE('',#38696,#38697,#31596,.T.);
#48352=EDGE_CURVE('',#38697,#38698,#20924,.T.);
#48353=EDGE_CURVE('',#38699,#38698,#31597,.T.);
#48354=EDGE_CURVE('',#38700,#38699,#31598,.T.);
#48355=EDGE_CURVE('',#38701,#38700,#31599,.T.);
#48356=EDGE_CURVE('',#38701,#38696,#20925,.T.);
#48357=EDGE_CURVE('',#38699,#38702,#20926,.T.);
#48358=EDGE_CURVE('',#38702,#38703,#31600,.T.);
#48359=EDGE_CURVE('',#38703,#38700,#20927,.T.);
#48360=EDGE_CURVE('',#38704,#38705,#31601,.T.);
#48361=EDGE_CURVE('',#38705,#38706,#20928,.T.);
#48362=EDGE_CURVE('',#38706,#38707,#31602,.T.);
#48363=EDGE_CURVE('',#38707,#38704,#20929,.T.);
#48364=EDGE_CURVE('',#38708,#38709,#31603,.T.);
#48365=EDGE_CURVE('',#38709,#38710,#20930,.T.);
#48366=EDGE_CURVE('',#38711,#38710,#31604,.T.);
#48367=EDGE_CURVE('',#38712,#38711,#31605,.T.);
#48368=EDGE_CURVE('',#38713,#38712,#31606,.T.);
#48369=EDGE_CURVE('',#38713,#38708,#20931,.T.);
#48370=EDGE_CURVE('',#38711,#38714,#20932,.T.);
#48371=EDGE_CURVE('',#38714,#38715,#31607,.T.);
#48372=EDGE_CURVE('',#38715,#38712,#20933,.T.);
#48373=EDGE_CURVE('',#37359,#38697,#31608,.T.);
#48374=EDGE_CURVE('',#38696,#37360,#31609,.T.);
#48375=EDGE_CURVE('',#38714,#36856,#680,.T.);
#48376=EDGE_CURVE('',#36855,#38715,#681,.T.);
#48377=EDGE_CURVE('',#38706,#38709,#682,.T.);
#48378=EDGE_CURVE('',#38708,#38707,#683,.T.);
#48379=EDGE_CURVE('',#38702,#38705,#684,.T.);
#48380=EDGE_CURVE('',#38704,#38703,#685,.T.);
#48381=EDGE_CURVE('',#38716,#38717,#31610,.T.);
#48382=EDGE_CURVE('',#38717,#38718,#20934,.T.);
#48383=EDGE_CURVE('',#38719,#38718,#31611,.T.);
#48384=EDGE_CURVE('',#38720,#38719,#31612,.T.);
#48385=EDGE_CURVE('',#38721,#38720,#31613,.T.);
#48386=EDGE_CURVE('',#38721,#38716,#20935,.T.);
#48387=EDGE_CURVE('',#38719,#38722,#20936,.T.);
#48388=EDGE_CURVE('',#38722,#38723,#31614,.T.);
#48389=EDGE_CURVE('',#38723,#38720,#20937,.T.);
#48390=EDGE_CURVE('',#38724,#38725,#31615,.T.);
#48391=EDGE_CURVE('',#38725,#38726,#20938,.T.);
#48392=EDGE_CURVE('',#38726,#38727,#31616,.T.);
#48393=EDGE_CURVE('',#38727,#38724,#20939,.T.);
#48394=EDGE_CURVE('',#38728,#38729,#31617,.T.);
#48395=EDGE_CURVE('',#38729,#38730,#20940,.T.);
#48396=EDGE_CURVE('',#38731,#38730,#31618,.T.);
#48397=EDGE_CURVE('',#38732,#38731,#31619,.T.);
#48398=EDGE_CURVE('',#38733,#38732,#31620,.T.);
#48399=EDGE_CURVE('',#38733,#38728,#20941,.T.);
#48400=EDGE_CURVE('',#38731,#38734,#20942,.T.);
#48401=EDGE_CURVE('',#38734,#38735,#31621,.T.);
#48402=EDGE_CURVE('',#38735,#38732,#20943,.T.);
#48403=EDGE_CURVE('',#37365,#38717,#31622,.T.);
#48404=EDGE_CURVE('',#38716,#37366,#31623,.T.);
#48405=EDGE_CURVE('',#38734,#36850,#686,.T.);
#48406=EDGE_CURVE('',#36849,#38735,#687,.T.);
#48407=EDGE_CURVE('',#38726,#38729,#688,.T.);
#48408=EDGE_CURVE('',#38728,#38727,#689,.T.);
#48409=EDGE_CURVE('',#38722,#38725,#690,.T.);
#48410=EDGE_CURVE('',#38724,#38723,#691,.T.);
#48411=EDGE_CURVE('',#38736,#38737,#31624,.T.);
#48412=EDGE_CURVE('',#38737,#38738,#20944,.T.);
#48413=EDGE_CURVE('',#38739,#38738,#31625,.T.);
#48414=EDGE_CURVE('',#38740,#38739,#31626,.T.);
#48415=EDGE_CURVE('',#38741,#38740,#31627,.T.);
#48416=EDGE_CURVE('',#38741,#38736,#20945,.T.);
#48417=EDGE_CURVE('',#38739,#38742,#20946,.T.);
#48418=EDGE_CURVE('',#38742,#38743,#31628,.T.);
#48419=EDGE_CURVE('',#38743,#38740,#20947,.T.);
#48420=EDGE_CURVE('',#38744,#38745,#31629,.T.);
#48421=EDGE_CURVE('',#38745,#38746,#20948,.T.);
#48422=EDGE_CURVE('',#38746,#38747,#31630,.T.);
#48423=EDGE_CURVE('',#38747,#38744,#20949,.T.);
#48424=EDGE_CURVE('',#38748,#38749,#31631,.T.);
#48425=EDGE_CURVE('',#38749,#38750,#20950,.T.);
#48426=EDGE_CURVE('',#38751,#38750,#31632,.T.);
#48427=EDGE_CURVE('',#38752,#38751,#31633,.T.);
#48428=EDGE_CURVE('',#38753,#38752,#31634,.T.);
#48429=EDGE_CURVE('',#38753,#38748,#20951,.T.);
#48430=EDGE_CURVE('',#38751,#38754,#20952,.T.);
#48431=EDGE_CURVE('',#38754,#38755,#31635,.T.);
#48432=EDGE_CURVE('',#38755,#38752,#20953,.T.);
#48433=EDGE_CURVE('',#37371,#38737,#31636,.T.);
#48434=EDGE_CURVE('',#38736,#37372,#31637,.T.);
#48435=EDGE_CURVE('',#38754,#36844,#692,.T.);
#48436=EDGE_CURVE('',#36843,#38755,#693,.T.);
#48437=EDGE_CURVE('',#38746,#38749,#694,.T.);
#48438=EDGE_CURVE('',#38748,#38747,#695,.T.);
#48439=EDGE_CURVE('',#38742,#38745,#696,.T.);
#48440=EDGE_CURVE('',#38744,#38743,#697,.T.);
#48441=EDGE_CURVE('',#38756,#38757,#20954,.T.);
#48442=EDGE_CURVE('',#38757,#38758,#31638,.T.);
#48443=EDGE_CURVE('',#38758,#38759,#20955,.T.);
#48444=EDGE_CURVE('',#38759,#38756,#31639,.T.);
#48445=EDGE_CURVE('',#38760,#38761,#698,.T.);
#48446=EDGE_CURVE('',#38761,#38762,#20956,.T.);
#48447=EDGE_CURVE('',#38762,#38763,#20957,.T.);
#48448=EDGE_CURVE('',#38763,#38764,#20958,.T.);
#48449=EDGE_CURVE('',#38764,#38765,#699,.T.);
#48450=EDGE_CURVE('',#38765,#38766,#20959,.T.);
#48451=EDGE_CURVE('',#38766,#38767,#20960,.T.);
#48452=EDGE_CURVE('',#38767,#38768,#700,.T.);
#48453=EDGE_CURVE('',#38768,#38769,#20961,.T.);
#48454=EDGE_CURVE('',#38769,#38770,#701,.T.);
#48455=EDGE_CURVE('',#38770,#38771,#20962,.T.);
#48456=EDGE_CURVE('',#38771,#38760,#20963,.T.);
#48457=EDGE_CURVE('',#38772,#38773,#702,.T.);
#48458=EDGE_CURVE('',#38773,#38774,#20964,.T.);
#48459=EDGE_CURVE('',#38774,#38775,#20965,.T.);
#48460=EDGE_CURVE('',#38775,#38776,#20966,.T.);
#48461=EDGE_CURVE('',#38776,#38777,#703,.T.);
#48462=EDGE_CURVE('',#38777,#38778,#20967,.T.);
#48463=EDGE_CURVE('',#38778,#38779,#20968,.T.);
#48464=EDGE_CURVE('',#38779,#38780,#704,.T.);
#48465=EDGE_CURVE('',#38780,#38781,#20969,.T.);
#48466=EDGE_CURVE('',#38781,#38782,#705,.T.);
#48467=EDGE_CURVE('',#38782,#38783,#20970,.T.);
#48468=EDGE_CURVE('',#38783,#38772,#20971,.T.);
#48469=EDGE_CURVE('',#38774,#38757,#4495,.T.);
#48470=EDGE_CURVE('',#38756,#38775,#4496,.T.);
#48471=EDGE_CURVE('',#38758,#38763,#4497,.T.);
#48472=EDGE_CURVE('',#38762,#38759,#4498,.T.);
#48473=EDGE_CURVE('',#38783,#38753,#706,.T.);
#48474=EDGE_CURVE('',#38748,#38782,#31640,.T.);
#48475=EDGE_CURVE('',#38747,#38781,#31641,.T.);
#48476=EDGE_CURVE('',#38772,#38755,#31642,.T.);
#48477=EDGE_CURVE('',#38744,#38780,#31643,.T.);
#48478=EDGE_CURVE('',#38773,#36843,#31644,.T.);
#48479=EDGE_CURVE('',#38743,#38779,#31645,.T.);
#48480=EDGE_CURVE('',#38774,#36842,#31646,.T.);
#48481=EDGE_CURVE('',#38741,#38778,#707,.T.);
#48482=EDGE_CURVE('',#38757,#36841,#31647,.T.);
#48483=EDGE_CURVE('',#38736,#38777,#31648,.T.);
#48484=EDGE_CURVE('',#38758,#36840,#31649,.T.);
#48485=EDGE_CURVE('',#37372,#38776,#31650,.T.);
#48486=EDGE_CURVE('',#38763,#37195,#31651,.T.);
#48487=EDGE_CURVE('',#37373,#38775,#31652,.T.);
#48488=EDGE_CURVE('',#38764,#37194,#31653,.T.);
#48489=EDGE_CURVE('',#37374,#38756,#31654,.T.);
#48490=EDGE_CURVE('',#38765,#37574,#31655,.T.);
#48491=EDGE_CURVE('',#37376,#38759,#31656,.T.);
#48492=EDGE_CURVE('',#38766,#37572,#708,.T.);
#48493=EDGE_CURVE('',#37377,#38762,#31657,.T.);
#48494=EDGE_CURVE('',#38767,#37571,#31658,.T.);
#48495=EDGE_CURVE('',#37378,#38761,#31659,.T.);
#48496=EDGE_CURVE('',#38768,#37564,#31660,.T.);
#48497=EDGE_CURVE('',#37559,#38760,#31661,.T.);
#48498=EDGE_CURVE('',#38769,#37567,#31662,.T.);
#48499=EDGE_CURVE('',#37560,#38771,#709,.T.);
#48500=EDGE_CURVE('',#38770,#37562,#31663,.T.);
#48501=EDGE_CURVE('',#38784,#38785,#20972,.T.);
#48502=EDGE_CURVE('',#38785,#38786,#31664,.T.);
#48503=EDGE_CURVE('',#38786,#38787,#20973,.T.);
#48504=EDGE_CURVE('',#38787,#38784,#31665,.T.);
#48505=EDGE_CURVE('',#38788,#38789,#710,.T.);
#48506=EDGE_CURVE('',#38789,#38790,#20974,.T.);
#48507=EDGE_CURVE('',#38790,#38791,#20975,.T.);
#48508=EDGE_CURVE('',#38791,#38792,#20976,.T.);
#48509=EDGE_CURVE('',#38792,#38793,#711,.T.);
#48510=EDGE_CURVE('',#38793,#38794,#20977,.T.);
#48511=EDGE_CURVE('',#38794,#38795,#20978,.T.);
#48512=EDGE_CURVE('',#38795,#38796,#712,.T.);
#48513=EDGE_CURVE('',#38796,#38797,#20979,.T.);
#48514=EDGE_CURVE('',#38797,#38798,#713,.T.);
#48515=EDGE_CURVE('',#38798,#38799,#20980,.T.);
#48516=EDGE_CURVE('',#38799,#38788,#20981,.T.);
#48517=EDGE_CURVE('',#38800,#38801,#714,.T.);
#48518=EDGE_CURVE('',#38801,#38802,#20982,.T.);
#48519=EDGE_CURVE('',#38802,#38803,#20983,.T.);
#48520=EDGE_CURVE('',#38803,#38804,#20984,.T.);
#48521=EDGE_CURVE('',#38804,#38805,#715,.T.);
#48522=EDGE_CURVE('',#38805,#38806,#20985,.T.);
#48523=EDGE_CURVE('',#38806,#38807,#20986,.T.);
#48524=EDGE_CURVE('',#38807,#38808,#716,.T.);
#48525=EDGE_CURVE('',#38808,#38809,#20987,.T.);
#48526=EDGE_CURVE('',#38809,#38810,#717,.T.);
#48527=EDGE_CURVE('',#38810,#38811,#20988,.T.);
#48528=EDGE_CURVE('',#38811,#38800,#20989,.T.);
#48529=EDGE_CURVE('',#38812,#38813,#20990,.T.);
#48530=EDGE_CURVE('',#38813,#38814,#31666,.T.);
#48531=EDGE_CURVE('',#38814,#38815,#20991,.T.);
#48532=EDGE_CURVE('',#38815,#38812,#31667,.T.);
#48533=EDGE_CURVE('',#38816,#38817,#718,.T.);
#48534=EDGE_CURVE('',#38817,#38818,#20992,.T.);
#48535=EDGE_CURVE('',#38818,#38819,#20993,.T.);
#48536=EDGE_CURVE('',#38819,#38820,#20994,.T.);
#48537=EDGE_CURVE('',#38820,#38821,#719,.T.);
#48538=EDGE_CURVE('',#38821,#38822,#20995,.T.);
#48539=EDGE_CURVE('',#38822,#38823,#20996,.T.);
#48540=EDGE_CURVE('',#38823,#38824,#720,.T.);
#48541=EDGE_CURVE('',#38824,#38825,#20997,.T.);
#48542=EDGE_CURVE('',#38825,#38826,#721,.T.);
#48543=EDGE_CURVE('',#38826,#38827,#20998,.T.);
#48544=EDGE_CURVE('',#38827,#38816,#20999,.T.);
#48545=EDGE_CURVE('',#38828,#38829,#722,.T.);
#48546=EDGE_CURVE('',#38829,#38830,#21000,.T.);
#48547=EDGE_CURVE('',#38830,#38831,#21001,.T.);
#48548=EDGE_CURVE('',#38831,#38832,#21002,.T.);
#48549=EDGE_CURVE('',#38832,#38833,#723,.T.);
#48550=EDGE_CURVE('',#38833,#38834,#21003,.T.);
#48551=EDGE_CURVE('',#38834,#38835,#21004,.T.);
#48552=EDGE_CURVE('',#38835,#38836,#724,.T.);
#48553=EDGE_CURVE('',#38836,#38837,#21005,.T.);
#48554=EDGE_CURVE('',#38837,#38838,#725,.T.);
#48555=EDGE_CURVE('',#38838,#38839,#21006,.T.);
#48556=EDGE_CURVE('',#38839,#38828,#21007,.T.);
#48557=EDGE_CURVE('',#38840,#38841,#21008,.T.);
#48558=EDGE_CURVE('',#38841,#38842,#31668,.T.);
#48559=EDGE_CURVE('',#38842,#38843,#21009,.T.);
#48560=EDGE_CURVE('',#38843,#38840,#31669,.T.);
#48561=EDGE_CURVE('',#38844,#38845,#726,.T.);
#48562=EDGE_CURVE('',#38845,#38846,#21010,.T.);
#48563=EDGE_CURVE('',#38846,#38847,#21011,.T.);
#48564=EDGE_CURVE('',#38847,#38848,#21012,.T.);
#48565=EDGE_CURVE('',#38848,#38849,#727,.T.);
#48566=EDGE_CURVE('',#38849,#38850,#21013,.T.);
#48567=EDGE_CURVE('',#38850,#38851,#21014,.T.);
#48568=EDGE_CURVE('',#38851,#38852,#728,.T.);
#48569=EDGE_CURVE('',#38852,#38853,#21015,.T.);
#48570=EDGE_CURVE('',#38853,#38854,#729,.T.);
#48571=EDGE_CURVE('',#38854,#38855,#21016,.T.);
#48572=EDGE_CURVE('',#38855,#38844,#21017,.T.);
#48573=EDGE_CURVE('',#38856,#38857,#730,.T.);
#48574=EDGE_CURVE('',#38857,#38858,#21018,.T.);
#48575=EDGE_CURVE('',#38858,#38859,#21019,.T.);
#48576=EDGE_CURVE('',#38859,#38860,#21020,.T.);
#48577=EDGE_CURVE('',#38860,#38861,#731,.T.);
#48578=EDGE_CURVE('',#38861,#38862,#21021,.T.);
#48579=EDGE_CURVE('',#38862,#38863,#21022,.T.);
#48580=EDGE_CURVE('',#38863,#38864,#732,.T.);
#48581=EDGE_CURVE('',#38864,#38865,#21023,.T.);
#48582=EDGE_CURVE('',#38865,#38866,#733,.T.);
#48583=EDGE_CURVE('',#38866,#38867,#21024,.T.);
#48584=EDGE_CURVE('',#38867,#38856,#21025,.T.);
#48585=EDGE_CURVE('',#38868,#38869,#21026,.T.);
#48586=EDGE_CURVE('',#38869,#38870,#31670,.T.);
#48587=EDGE_CURVE('',#38870,#38871,#21027,.T.);
#48588=EDGE_CURVE('',#38871,#38868,#31671,.T.);
#48589=EDGE_CURVE('',#38872,#38873,#734,.T.);
#48590=EDGE_CURVE('',#38873,#38874,#21028,.T.);
#48591=EDGE_CURVE('',#38874,#38875,#21029,.T.);
#48592=EDGE_CURVE('',#38875,#38876,#21030,.T.);
#48593=EDGE_CURVE('',#38876,#38877,#735,.T.);
#48594=EDGE_CURVE('',#38877,#38878,#21031,.T.);
#48595=EDGE_CURVE('',#38878,#38879,#21032,.T.);
#48596=EDGE_CURVE('',#38879,#38880,#736,.T.);
#48597=EDGE_CURVE('',#38880,#38881,#21033,.T.);
#48598=EDGE_CURVE('',#38881,#38882,#737,.T.);
#48599=EDGE_CURVE('',#38882,#38883,#21034,.T.);
#48600=EDGE_CURVE('',#38883,#38872,#21035,.T.);
#48601=EDGE_CURVE('',#38884,#38885,#738,.T.);
#48602=EDGE_CURVE('',#38885,#38886,#21036,.T.);
#48603=EDGE_CURVE('',#38886,#38887,#21037,.T.);
#48604=EDGE_CURVE('',#38887,#38888,#21038,.T.);
#48605=EDGE_CURVE('',#38888,#38889,#739,.T.);
#48606=EDGE_CURVE('',#38889,#38890,#21039,.T.);
#48607=EDGE_CURVE('',#38890,#38891,#21040,.T.);
#48608=EDGE_CURVE('',#38891,#38892,#740,.T.);
#48609=EDGE_CURVE('',#38892,#38893,#21041,.T.);
#48610=EDGE_CURVE('',#38893,#38894,#741,.T.);
#48611=EDGE_CURVE('',#38894,#38895,#21042,.T.);
#48612=EDGE_CURVE('',#38895,#38884,#21043,.T.);
#48613=EDGE_CURVE('',#38896,#38897,#21044,.T.);
#48614=EDGE_CURVE('',#38897,#38898,#31672,.T.);
#48615=EDGE_CURVE('',#38898,#38899,#21045,.T.);
#48616=EDGE_CURVE('',#38899,#38896,#31673,.T.);
#48617=EDGE_CURVE('',#38900,#38901,#742,.T.);
#48618=EDGE_CURVE('',#38901,#38902,#21046,.T.);
#48619=EDGE_CURVE('',#38902,#38903,#21047,.T.);
#48620=EDGE_CURVE('',#38903,#38904,#21048,.T.);
#48621=EDGE_CURVE('',#38904,#38905,#743,.T.);
#48622=EDGE_CURVE('',#38905,#38906,#21049,.T.);
#48623=EDGE_CURVE('',#38906,#38907,#21050,.T.);
#48624=EDGE_CURVE('',#38907,#38908,#744,.T.);
#48625=EDGE_CURVE('',#38908,#38909,#21051,.T.);
#48626=EDGE_CURVE('',#38909,#38910,#745,.T.);
#48627=EDGE_CURVE('',#38910,#38911,#21052,.T.);
#48628=EDGE_CURVE('',#38911,#38900,#21053,.T.);
#48629=EDGE_CURVE('',#38912,#38913,#746,.T.);
#48630=EDGE_CURVE('',#38913,#38914,#21054,.T.);
#48631=EDGE_CURVE('',#38914,#38915,#21055,.T.);
#48632=EDGE_CURVE('',#38915,#38916,#21056,.T.);
#48633=EDGE_CURVE('',#38916,#38917,#747,.T.);
#48634=EDGE_CURVE('',#38917,#38918,#21057,.T.);
#48635=EDGE_CURVE('',#38918,#38919,#21058,.T.);
#48636=EDGE_CURVE('',#38919,#38920,#748,.T.);
#48637=EDGE_CURVE('',#38920,#38921,#21059,.T.);
#48638=EDGE_CURVE('',#38921,#38922,#749,.T.);
#48639=EDGE_CURVE('',#38922,#38923,#21060,.T.);
#48640=EDGE_CURVE('',#38923,#38912,#21061,.T.);
#48641=EDGE_CURVE('',#38924,#38925,#21062,.T.);
#48642=EDGE_CURVE('',#38925,#38926,#31674,.T.);
#48643=EDGE_CURVE('',#38926,#38927,#21063,.T.);
#48644=EDGE_CURVE('',#38927,#38924,#31675,.T.);
#48645=EDGE_CURVE('',#38928,#38929,#750,.T.);
#48646=EDGE_CURVE('',#38929,#38930,#21064,.T.);
#48647=EDGE_CURVE('',#38930,#38931,#21065,.T.);
#48648=EDGE_CURVE('',#38931,#38932,#21066,.T.);
#48649=EDGE_CURVE('',#38932,#38933,#751,.T.);
#48650=EDGE_CURVE('',#38933,#38934,#21067,.T.);
#48651=EDGE_CURVE('',#38934,#38935,#21068,.T.);
#48652=EDGE_CURVE('',#38935,#38936,#752,.T.);
#48653=EDGE_CURVE('',#38936,#38937,#21069,.T.);
#48654=EDGE_CURVE('',#38937,#38938,#753,.T.);
#48655=EDGE_CURVE('',#38938,#38939,#21070,.T.);
#48656=EDGE_CURVE('',#38939,#38928,#21071,.T.);
#48657=EDGE_CURVE('',#38940,#38941,#754,.T.);
#48658=EDGE_CURVE('',#38941,#38942,#21072,.T.);
#48659=EDGE_CURVE('',#38942,#38943,#21073,.T.);
#48660=EDGE_CURVE('',#38943,#38944,#21074,.T.);
#48661=EDGE_CURVE('',#38944,#38945,#755,.T.);
#48662=EDGE_CURVE('',#38945,#38946,#21075,.T.);
#48663=EDGE_CURVE('',#38946,#38947,#21076,.T.);
#48664=EDGE_CURVE('',#38947,#38948,#756,.T.);
#48665=EDGE_CURVE('',#38948,#38949,#21077,.T.);
#48666=EDGE_CURVE('',#38949,#38950,#757,.T.);
#48667=EDGE_CURVE('',#38950,#38951,#21078,.T.);
#48668=EDGE_CURVE('',#38951,#38940,#21079,.T.);
#48669=EDGE_CURVE('',#38952,#38953,#21080,.T.);
#48670=EDGE_CURVE('',#38953,#38954,#31676,.T.);
#48671=EDGE_CURVE('',#38954,#38955,#21081,.T.);
#48672=EDGE_CURVE('',#38955,#38952,#31677,.T.);
#48673=EDGE_CURVE('',#38956,#38957,#758,.T.);
#48674=EDGE_CURVE('',#38957,#38958,#21082,.T.);
#48675=EDGE_CURVE('',#38958,#38959,#21083,.T.);
#48676=EDGE_CURVE('',#38959,#38960,#21084,.T.);
#48677=EDGE_CURVE('',#38960,#38961,#759,.T.);
#48678=EDGE_CURVE('',#38961,#38962,#21085,.T.);
#48679=EDGE_CURVE('',#38962,#38963,#21086,.T.);
#48680=EDGE_CURVE('',#38963,#38964,#760,.T.);
#48681=EDGE_CURVE('',#38964,#38965,#21087,.T.);
#48682=EDGE_CURVE('',#38965,#38966,#761,.T.);
#48683=EDGE_CURVE('',#38966,#38967,#21088,.T.);
#48684=EDGE_CURVE('',#38967,#38956,#21089,.T.);
#48685=EDGE_CURVE('',#38968,#38969,#762,.T.);
#48686=EDGE_CURVE('',#38969,#38970,#21090,.T.);
#48687=EDGE_CURVE('',#38970,#38971,#21091,.T.);
#48688=EDGE_CURVE('',#38971,#38972,#21092,.T.);
#48689=EDGE_CURVE('',#38972,#38973,#763,.T.);
#48690=EDGE_CURVE('',#38973,#38974,#21093,.T.);
#48691=EDGE_CURVE('',#38974,#38975,#21094,.T.);
#48692=EDGE_CURVE('',#38975,#38976,#764,.T.);
#48693=EDGE_CURVE('',#38976,#38977,#21095,.T.);
#48694=EDGE_CURVE('',#38977,#38978,#765,.T.);
#48695=EDGE_CURVE('',#38978,#38979,#21096,.T.);
#48696=EDGE_CURVE('',#38979,#38968,#21097,.T.);
#48697=EDGE_CURVE('',#38980,#38981,#21098,.T.);
#48698=EDGE_CURVE('',#38981,#38982,#31678,.T.);
#48699=EDGE_CURVE('',#38982,#38983,#21099,.T.);
#48700=EDGE_CURVE('',#38983,#38980,#31679,.T.);
#48701=EDGE_CURVE('',#38984,#38985,#766,.T.);
#48702=EDGE_CURVE('',#38985,#38986,#21100,.T.);
#48703=EDGE_CURVE('',#38986,#38987,#21101,.T.);
#48704=EDGE_CURVE('',#38987,#38988,#21102,.T.);
#48705=EDGE_CURVE('',#38988,#38989,#767,.T.);
#48706=EDGE_CURVE('',#38989,#38990,#21103,.T.);
#48707=EDGE_CURVE('',#38990,#38991,#21104,.T.);
#48708=EDGE_CURVE('',#38991,#38992,#768,.T.);
#48709=EDGE_CURVE('',#38992,#38993,#21105,.T.);
#48710=EDGE_CURVE('',#38993,#38994,#769,.T.);
#48711=EDGE_CURVE('',#38994,#38995,#21106,.T.);
#48712=EDGE_CURVE('',#38995,#38984,#21107,.T.);
#48713=EDGE_CURVE('',#38996,#38997,#770,.T.);
#48714=EDGE_CURVE('',#38997,#38998,#21108,.T.);
#48715=EDGE_CURVE('',#38998,#38999,#21109,.T.);
#48716=EDGE_CURVE('',#38999,#39000,#21110,.T.);
#48717=EDGE_CURVE('',#39000,#39001,#771,.T.);
#48718=EDGE_CURVE('',#39001,#39002,#21111,.T.);
#48719=EDGE_CURVE('',#39002,#39003,#21112,.T.);
#48720=EDGE_CURVE('',#39003,#39004,#772,.T.);
#48721=EDGE_CURVE('',#39004,#39005,#21113,.T.);
#48722=EDGE_CURVE('',#39005,#39006,#773,.T.);
#48723=EDGE_CURVE('',#39006,#39007,#21114,.T.);
#48724=EDGE_CURVE('',#39007,#38996,#21115,.T.);
#48725=EDGE_CURVE('',#39008,#39009,#21116,.T.);
#48726=EDGE_CURVE('',#39009,#39010,#31680,.T.);
#48727=EDGE_CURVE('',#39010,#39011,#21117,.T.);
#48728=EDGE_CURVE('',#39011,#39008,#31681,.T.);
#48729=EDGE_CURVE('',#39012,#39013,#774,.T.);
#48730=EDGE_CURVE('',#39013,#39014,#21118,.T.);
#48731=EDGE_CURVE('',#39014,#39015,#21119,.T.);
#48732=EDGE_CURVE('',#39015,#39016,#21120,.T.);
#48733=EDGE_CURVE('',#39016,#39017,#775,.T.);
#48734=EDGE_CURVE('',#39017,#39018,#21121,.T.);
#48735=EDGE_CURVE('',#39018,#39019,#21122,.T.);
#48736=EDGE_CURVE('',#39019,#39020,#776,.T.);
#48737=EDGE_CURVE('',#39020,#39021,#21123,.T.);
#48738=EDGE_CURVE('',#39021,#39022,#777,.T.);
#48739=EDGE_CURVE('',#39022,#39023,#21124,.T.);
#48740=EDGE_CURVE('',#39023,#39012,#21125,.T.);
#48741=EDGE_CURVE('',#39024,#39025,#778,.T.);
#48742=EDGE_CURVE('',#39025,#39026,#21126,.T.);
#48743=EDGE_CURVE('',#39026,#39027,#21127,.T.);
#48744=EDGE_CURVE('',#39027,#39028,#21128,.T.);
#48745=EDGE_CURVE('',#39028,#39029,#779,.T.);
#48746=EDGE_CURVE('',#39029,#39030,#21129,.T.);
#48747=EDGE_CURVE('',#39030,#39031,#21130,.T.);
#48748=EDGE_CURVE('',#39031,#39032,#780,.T.);
#48749=EDGE_CURVE('',#39032,#39033,#21131,.T.);
#48750=EDGE_CURVE('',#39033,#39034,#781,.T.);
#48751=EDGE_CURVE('',#39034,#39035,#21132,.T.);
#48752=EDGE_CURVE('',#39035,#39024,#21133,.T.);
#48753=EDGE_CURVE('',#39036,#39037,#21134,.T.);
#48754=EDGE_CURVE('',#39037,#39038,#31682,.T.);
#48755=EDGE_CURVE('',#39038,#39039,#21135,.T.);
#48756=EDGE_CURVE('',#39039,#39036,#31683,.T.);
#48757=EDGE_CURVE('',#39040,#39041,#782,.T.);
#48758=EDGE_CURVE('',#39041,#39042,#21136,.T.);
#48759=EDGE_CURVE('',#39042,#39043,#21137,.T.);
#48760=EDGE_CURVE('',#39043,#39044,#21138,.T.);
#48761=EDGE_CURVE('',#39044,#39045,#783,.T.);
#48762=EDGE_CURVE('',#39045,#39046,#21139,.T.);
#48763=EDGE_CURVE('',#39046,#39047,#21140,.T.);
#48764=EDGE_CURVE('',#39047,#39048,#784,.T.);
#48765=EDGE_CURVE('',#39048,#39049,#21141,.T.);
#48766=EDGE_CURVE('',#39049,#39050,#785,.T.);
#48767=EDGE_CURVE('',#39050,#39051,#21142,.T.);
#48768=EDGE_CURVE('',#39051,#39040,#21143,.T.);
#48769=EDGE_CURVE('',#39052,#39053,#786,.T.);
#48770=EDGE_CURVE('',#39053,#39054,#21144,.T.);
#48771=EDGE_CURVE('',#39054,#39055,#21145,.T.);
#48772=EDGE_CURVE('',#39055,#39056,#21146,.T.);
#48773=EDGE_CURVE('',#39056,#39057,#787,.T.);
#48774=EDGE_CURVE('',#39057,#39058,#21147,.T.);
#48775=EDGE_CURVE('',#39058,#39059,#21148,.T.);
#48776=EDGE_CURVE('',#39059,#39060,#788,.T.);
#48777=EDGE_CURVE('',#39060,#39061,#21149,.T.);
#48778=EDGE_CURVE('',#39061,#39062,#789,.T.);
#48779=EDGE_CURVE('',#39062,#39063,#21150,.T.);
#48780=EDGE_CURVE('',#39063,#39052,#21151,.T.);
#48781=EDGE_CURVE('',#39064,#39065,#21152,.T.);
#48782=EDGE_CURVE('',#39065,#39066,#31684,.T.);
#48783=EDGE_CURVE('',#39066,#39067,#21153,.T.);
#48784=EDGE_CURVE('',#39067,#39064,#31685,.T.);
#48785=EDGE_CURVE('',#39068,#39069,#790,.T.);
#48786=EDGE_CURVE('',#39069,#39070,#21154,.T.);
#48787=EDGE_CURVE('',#39070,#39071,#21155,.T.);
#48788=EDGE_CURVE('',#39071,#39072,#21156,.T.);
#48789=EDGE_CURVE('',#39072,#39073,#791,.T.);
#48790=EDGE_CURVE('',#39073,#39074,#21157,.T.);
#48791=EDGE_CURVE('',#39074,#39075,#21158,.T.);
#48792=EDGE_CURVE('',#39075,#39076,#792,.T.);
#48793=EDGE_CURVE('',#39076,#39077,#21159,.T.);
#48794=EDGE_CURVE('',#39077,#39078,#793,.T.);
#48795=EDGE_CURVE('',#39078,#39079,#21160,.T.);
#48796=EDGE_CURVE('',#39079,#39068,#21161,.T.);
#48797=EDGE_CURVE('',#39080,#39081,#794,.T.);
#48798=EDGE_CURVE('',#39081,#39082,#21162,.T.);
#48799=EDGE_CURVE('',#39082,#39083,#21163,.T.);
#48800=EDGE_CURVE('',#39083,#39084,#21164,.T.);
#48801=EDGE_CURVE('',#39084,#39085,#795,.T.);
#48802=EDGE_CURVE('',#39085,#39086,#21165,.T.);
#48803=EDGE_CURVE('',#39086,#39087,#21166,.T.);
#48804=EDGE_CURVE('',#39087,#39088,#796,.T.);
#48805=EDGE_CURVE('',#39088,#39089,#21167,.T.);
#48806=EDGE_CURVE('',#39089,#39090,#797,.T.);
#48807=EDGE_CURVE('',#39090,#39091,#21168,.T.);
#48808=EDGE_CURVE('',#39091,#39080,#21169,.T.);
#48809=EDGE_CURVE('',#39092,#39093,#21170,.T.);
#48810=EDGE_CURVE('',#39093,#39094,#31686,.T.);
#48811=EDGE_CURVE('',#39094,#39095,#21171,.T.);
#48812=EDGE_CURVE('',#39095,#39092,#31687,.T.);
#48813=EDGE_CURVE('',#39096,#39097,#798,.T.);
#48814=EDGE_CURVE('',#39097,#39098,#21172,.T.);
#48815=EDGE_CURVE('',#39098,#39099,#21173,.T.);
#48816=EDGE_CURVE('',#39099,#39100,#21174,.T.);
#48817=EDGE_CURVE('',#39100,#39101,#799,.T.);
#48818=EDGE_CURVE('',#39101,#39102,#21175,.T.);
#48819=EDGE_CURVE('',#39102,#39103,#21176,.T.);
#48820=EDGE_CURVE('',#39103,#39104,#800,.T.);
#48821=EDGE_CURVE('',#39104,#39105,#21177,.T.);
#48822=EDGE_CURVE('',#39105,#39106,#801,.T.);
#48823=EDGE_CURVE('',#39106,#39107,#21178,.T.);
#48824=EDGE_CURVE('',#39107,#39096,#21179,.T.);
#48825=EDGE_CURVE('',#39108,#39109,#802,.T.);
#48826=EDGE_CURVE('',#39109,#39110,#21180,.T.);
#48827=EDGE_CURVE('',#39110,#39111,#21181,.T.);
#48828=EDGE_CURVE('',#39111,#39112,#21182,.T.);
#48829=EDGE_CURVE('',#39112,#39113,#803,.T.);
#48830=EDGE_CURVE('',#39113,#39114,#21183,.T.);
#48831=EDGE_CURVE('',#39114,#39115,#21184,.T.);
#48832=EDGE_CURVE('',#39115,#39116,#804,.T.);
#48833=EDGE_CURVE('',#39116,#39117,#21185,.T.);
#48834=EDGE_CURVE('',#39117,#39118,#805,.T.);
#48835=EDGE_CURVE('',#39118,#39119,#21186,.T.);
#48836=EDGE_CURVE('',#39119,#39108,#21187,.T.);
#48837=EDGE_CURVE('',#39120,#39121,#21188,.T.);
#48838=EDGE_CURVE('',#39121,#39122,#31688,.T.);
#48839=EDGE_CURVE('',#39122,#39123,#21189,.T.);
#48840=EDGE_CURVE('',#39123,#39120,#31689,.T.);
#48841=EDGE_CURVE('',#39124,#39125,#806,.T.);
#48842=EDGE_CURVE('',#39125,#39126,#21190,.T.);
#48843=EDGE_CURVE('',#39126,#39127,#21191,.T.);
#48844=EDGE_CURVE('',#39127,#39128,#21192,.T.);
#48845=EDGE_CURVE('',#39128,#39129,#807,.T.);
#48846=EDGE_CURVE('',#39129,#39130,#21193,.T.);
#48847=EDGE_CURVE('',#39130,#39131,#21194,.T.);
#48848=EDGE_CURVE('',#39131,#39132,#808,.T.);
#48849=EDGE_CURVE('',#39132,#39133,#21195,.T.);
#48850=EDGE_CURVE('',#39133,#39134,#809,.T.);
#48851=EDGE_CURVE('',#39134,#39135,#21196,.T.);
#48852=EDGE_CURVE('',#39135,#39124,#21197,.T.);
#48853=EDGE_CURVE('',#39136,#39137,#810,.T.);
#48854=EDGE_CURVE('',#39137,#39138,#21198,.T.);
#48855=EDGE_CURVE('',#39138,#39139,#21199,.T.);
#48856=EDGE_CURVE('',#39139,#39140,#21200,.T.);
#48857=EDGE_CURVE('',#39140,#39141,#811,.T.);
#48858=EDGE_CURVE('',#39141,#39142,#21201,.T.);
#48859=EDGE_CURVE('',#39142,#39143,#21202,.T.);
#48860=EDGE_CURVE('',#39143,#39144,#812,.T.);
#48861=EDGE_CURVE('',#39144,#39145,#21203,.T.);
#48862=EDGE_CURVE('',#39145,#39146,#813,.T.);
#48863=EDGE_CURVE('',#39146,#39147,#21204,.T.);
#48864=EDGE_CURVE('',#39147,#39136,#21205,.T.);
#48865=EDGE_CURVE('',#39148,#39149,#21206,.T.);
#48866=EDGE_CURVE('',#39149,#39150,#31690,.T.);
#48867=EDGE_CURVE('',#39150,#39151,#21207,.T.);
#48868=EDGE_CURVE('',#39151,#39148,#31691,.T.);
#48869=EDGE_CURVE('',#39152,#39153,#814,.T.);
#48870=EDGE_CURVE('',#39153,#39154,#21208,.T.);
#48871=EDGE_CURVE('',#39154,#39155,#21209,.T.);
#48872=EDGE_CURVE('',#39155,#39156,#21210,.T.);
#48873=EDGE_CURVE('',#39156,#39157,#815,.T.);
#48874=EDGE_CURVE('',#39157,#39158,#21211,.T.);
#48875=EDGE_CURVE('',#39158,#39159,#21212,.T.);
#48876=EDGE_CURVE('',#39159,#39160,#816,.T.);
#48877=EDGE_CURVE('',#39160,#39161,#21213,.T.);
#48878=EDGE_CURVE('',#39161,#39162,#817,.T.);
#48879=EDGE_CURVE('',#39162,#39163,#21214,.T.);
#48880=EDGE_CURVE('',#39163,#39152,#21215,.T.);
#48881=EDGE_CURVE('',#39164,#39165,#818,.T.);
#48882=EDGE_CURVE('',#39165,#39166,#21216,.T.);
#48883=EDGE_CURVE('',#39166,#39167,#21217,.T.);
#48884=EDGE_CURVE('',#39167,#39168,#21218,.T.);
#48885=EDGE_CURVE('',#39168,#39169,#819,.T.);
#48886=EDGE_CURVE('',#39169,#39170,#21219,.T.);
#48887=EDGE_CURVE('',#39170,#39171,#21220,.T.);
#48888=EDGE_CURVE('',#39171,#39172,#820,.T.);
#48889=EDGE_CURVE('',#39172,#39173,#21221,.T.);
#48890=EDGE_CURVE('',#39173,#39174,#821,.T.);
#48891=EDGE_CURVE('',#39174,#39175,#21222,.T.);
#48892=EDGE_CURVE('',#39175,#39164,#21223,.T.);
#48893=EDGE_CURVE('',#39176,#39177,#21224,.T.);
#48894=EDGE_CURVE('',#39177,#39178,#31692,.T.);
#48895=EDGE_CURVE('',#39178,#39179,#21225,.T.);
#48896=EDGE_CURVE('',#39179,#39176,#31693,.T.);
#48897=EDGE_CURVE('',#39180,#39181,#822,.T.);
#48898=EDGE_CURVE('',#39181,#39182,#21226,.T.);
#48899=EDGE_CURVE('',#39182,#39183,#21227,.T.);
#48900=EDGE_CURVE('',#39183,#39184,#21228,.T.);
#48901=EDGE_CURVE('',#39184,#39185,#823,.T.);
#48902=EDGE_CURVE('',#39185,#39186,#21229,.T.);
#48903=EDGE_CURVE('',#39186,#39187,#21230,.T.);
#48904=EDGE_CURVE('',#39187,#39188,#824,.T.);
#48905=EDGE_CURVE('',#39188,#39189,#21231,.T.);
#48906=EDGE_CURVE('',#39189,#39190,#825,.T.);
#48907=EDGE_CURVE('',#39190,#39191,#21232,.T.);
#48908=EDGE_CURVE('',#39191,#39180,#21233,.T.);
#48909=EDGE_CURVE('',#39192,#39193,#826,.T.);
#48910=EDGE_CURVE('',#39193,#39194,#21234,.T.);
#48911=EDGE_CURVE('',#39194,#39195,#21235,.T.);
#48912=EDGE_CURVE('',#39195,#39196,#21236,.T.);
#48913=EDGE_CURVE('',#39196,#39197,#827,.T.);
#48914=EDGE_CURVE('',#39197,#39198,#21237,.T.);
#48915=EDGE_CURVE('',#39198,#39199,#21238,.T.);
#48916=EDGE_CURVE('',#39199,#39200,#828,.T.);
#48917=EDGE_CURVE('',#39200,#39201,#21239,.T.);
#48918=EDGE_CURVE('',#39201,#39202,#829,.T.);
#48919=EDGE_CURVE('',#39202,#39203,#21240,.T.);
#48920=EDGE_CURVE('',#39203,#39192,#21241,.T.);
#48921=EDGE_CURVE('',#39204,#39205,#21242,.T.);
#48922=EDGE_CURVE('',#39205,#39206,#31694,.T.);
#48923=EDGE_CURVE('',#39206,#39207,#21243,.T.);
#48924=EDGE_CURVE('',#39207,#39204,#31695,.T.);
#48925=EDGE_CURVE('',#39208,#39209,#830,.T.);
#48926=EDGE_CURVE('',#39209,#39210,#21244,.T.);
#48927=EDGE_CURVE('',#39210,#39211,#21245,.T.);
#48928=EDGE_CURVE('',#39211,#39212,#21246,.T.);
#48929=EDGE_CURVE('',#39212,#39213,#831,.T.);
#48930=EDGE_CURVE('',#39213,#39214,#21247,.T.);
#48931=EDGE_CURVE('',#39214,#39215,#21248,.T.);
#48932=EDGE_CURVE('',#39215,#39216,#832,.T.);
#48933=EDGE_CURVE('',#39216,#39217,#21249,.T.);
#48934=EDGE_CURVE('',#39217,#39218,#833,.T.);
#48935=EDGE_CURVE('',#39218,#39219,#21250,.T.);
#48936=EDGE_CURVE('',#39219,#39208,#21251,.T.);
#48937=EDGE_CURVE('',#39220,#39221,#834,.T.);
#48938=EDGE_CURVE('',#39221,#39222,#21252,.T.);
#48939=EDGE_CURVE('',#39222,#39223,#21253,.T.);
#48940=EDGE_CURVE('',#39223,#39224,#21254,.T.);
#48941=EDGE_CURVE('',#39224,#39225,#835,.T.);
#48942=EDGE_CURVE('',#39225,#39226,#21255,.T.);
#48943=EDGE_CURVE('',#39226,#39227,#21256,.T.);
#48944=EDGE_CURVE('',#39227,#39228,#836,.T.);
#48945=EDGE_CURVE('',#39228,#39229,#21257,.T.);
#48946=EDGE_CURVE('',#39229,#39230,#837,.T.);
#48947=EDGE_CURVE('',#39230,#39231,#21258,.T.);
#48948=EDGE_CURVE('',#39231,#39220,#21259,.T.);
#48949=EDGE_CURVE('',#39232,#39233,#21260,.T.);
#48950=EDGE_CURVE('',#39233,#39234,#31696,.T.);
#48951=EDGE_CURVE('',#39234,#39235,#21261,.T.);
#48952=EDGE_CURVE('',#39235,#39232,#31697,.T.);
#48953=EDGE_CURVE('',#39236,#39237,#838,.T.);
#48954=EDGE_CURVE('',#39237,#39238,#21262,.T.);
#48955=EDGE_CURVE('',#39238,#39239,#21263,.T.);
#48956=EDGE_CURVE('',#39239,#39240,#21264,.T.);
#48957=EDGE_CURVE('',#39240,#39241,#839,.T.);
#48958=EDGE_CURVE('',#39241,#39242,#21265,.T.);
#48959=EDGE_CURVE('',#39242,#39243,#21266,.T.);
#48960=EDGE_CURVE('',#39243,#39244,#840,.T.);
#48961=EDGE_CURVE('',#39244,#39245,#21267,.T.);
#48962=EDGE_CURVE('',#39245,#39246,#841,.T.);
#48963=EDGE_CURVE('',#39246,#39247,#21268,.T.);
#48964=EDGE_CURVE('',#39247,#39236,#21269,.T.);
#48965=EDGE_CURVE('',#39248,#39249,#842,.T.);
#48966=EDGE_CURVE('',#39249,#39250,#21270,.T.);
#48967=EDGE_CURVE('',#39250,#39251,#21271,.T.);
#48968=EDGE_CURVE('',#39251,#39252,#21272,.T.);
#48969=EDGE_CURVE('',#39252,#39253,#843,.T.);
#48970=EDGE_CURVE('',#39253,#39254,#21273,.T.);
#48971=EDGE_CURVE('',#39254,#39255,#21274,.T.);
#48972=EDGE_CURVE('',#39255,#39256,#844,.T.);
#48973=EDGE_CURVE('',#39256,#39257,#21275,.T.);
#48974=EDGE_CURVE('',#39257,#39258,#845,.T.);
#48975=EDGE_CURVE('',#39258,#39259,#21276,.T.);
#48976=EDGE_CURVE('',#39259,#39248,#21277,.T.);
#48977=EDGE_CURVE('',#39260,#39261,#21278,.T.);
#48978=EDGE_CURVE('',#39261,#39262,#31698,.T.);
#48979=EDGE_CURVE('',#39262,#39263,#21279,.T.);
#48980=EDGE_CURVE('',#39263,#39260,#31699,.T.);
#48981=EDGE_CURVE('',#39264,#39265,#846,.T.);
#48982=EDGE_CURVE('',#39265,#39266,#21280,.T.);
#48983=EDGE_CURVE('',#39266,#39267,#21281,.T.);
#48984=EDGE_CURVE('',#39267,#39268,#21282,.T.);
#48985=EDGE_CURVE('',#39268,#39269,#847,.T.);
#48986=EDGE_CURVE('',#39269,#39270,#21283,.T.);
#48987=EDGE_CURVE('',#39270,#39271,#21284,.T.);
#48988=EDGE_CURVE('',#39271,#39272,#848,.T.);
#48989=EDGE_CURVE('',#39272,#39273,#21285,.T.);
#48990=EDGE_CURVE('',#39273,#39274,#849,.T.);
#48991=EDGE_CURVE('',#39274,#39275,#21286,.T.);
#48992=EDGE_CURVE('',#39275,#39264,#21287,.T.);
#48993=EDGE_CURVE('',#39276,#39277,#850,.T.);
#48994=EDGE_CURVE('',#39277,#39278,#21288,.T.);
#48995=EDGE_CURVE('',#39278,#39279,#21289,.T.);
#48996=EDGE_CURVE('',#39279,#39280,#21290,.T.);
#48997=EDGE_CURVE('',#39280,#39281,#851,.T.);
#48998=EDGE_CURVE('',#39281,#39282,#21291,.T.);
#48999=EDGE_CURVE('',#39282,#39283,#21292,.T.);
#49000=EDGE_CURVE('',#39283,#39284,#852,.T.);
#49001=EDGE_CURVE('',#39284,#39285,#21293,.T.);
#49002=EDGE_CURVE('',#39285,#39286,#853,.T.);
#49003=EDGE_CURVE('',#39286,#39287,#21294,.T.);
#49004=EDGE_CURVE('',#39287,#39276,#21295,.T.);
#49005=EDGE_CURVE('',#39288,#39289,#21296,.T.);
#49006=EDGE_CURVE('',#39289,#39290,#31700,.T.);
#49007=EDGE_CURVE('',#39290,#39291,#21297,.T.);
#49008=EDGE_CURVE('',#39291,#39288,#31701,.T.);
#49009=EDGE_CURVE('',#39292,#39293,#854,.T.);
#49010=EDGE_CURVE('',#39293,#39294,#21298,.T.);
#49011=EDGE_CURVE('',#39294,#39295,#21299,.T.);
#49012=EDGE_CURVE('',#39295,#39296,#21300,.T.);
#49013=EDGE_CURVE('',#39296,#39297,#855,.T.);
#49014=EDGE_CURVE('',#39297,#39298,#21301,.T.);
#49015=EDGE_CURVE('',#39298,#39299,#21302,.T.);
#49016=EDGE_CURVE('',#39299,#39300,#856,.T.);
#49017=EDGE_CURVE('',#39300,#39301,#21303,.T.);
#49018=EDGE_CURVE('',#39301,#39302,#857,.T.);
#49019=EDGE_CURVE('',#39302,#39303,#21304,.T.);
#49020=EDGE_CURVE('',#39303,#39292,#21305,.T.);
#49021=EDGE_CURVE('',#39304,#39305,#858,.T.);
#49022=EDGE_CURVE('',#39305,#39306,#21306,.T.);
#49023=EDGE_CURVE('',#39306,#39307,#21307,.T.);
#49024=EDGE_CURVE('',#39307,#39308,#21308,.T.);
#49025=EDGE_CURVE('',#39308,#39309,#859,.T.);
#49026=EDGE_CURVE('',#39309,#39310,#21309,.T.);
#49027=EDGE_CURVE('',#39310,#39311,#21310,.T.);
#49028=EDGE_CURVE('',#39311,#39312,#860,.T.);
#49029=EDGE_CURVE('',#39312,#39313,#21311,.T.);
#49030=EDGE_CURVE('',#39313,#39314,#861,.T.);
#49031=EDGE_CURVE('',#39314,#39315,#21312,.T.);
#49032=EDGE_CURVE('',#39315,#39304,#21313,.T.);
#49033=EDGE_CURVE('',#39316,#39317,#21314,.T.);
#49034=EDGE_CURVE('',#39317,#39318,#31702,.T.);
#49035=EDGE_CURVE('',#39318,#39319,#21315,.T.);
#49036=EDGE_CURVE('',#39319,#39316,#31703,.T.);
#49037=EDGE_CURVE('',#39320,#39321,#862,.T.);
#49038=EDGE_CURVE('',#39321,#39322,#21316,.T.);
#49039=EDGE_CURVE('',#39322,#39323,#21317,.T.);
#49040=EDGE_CURVE('',#39323,#39324,#21318,.T.);
#49041=EDGE_CURVE('',#39324,#39325,#863,.T.);
#49042=EDGE_CURVE('',#39325,#39326,#21319,.T.);
#49043=EDGE_CURVE('',#39326,#39327,#21320,.T.);
#49044=EDGE_CURVE('',#39327,#39328,#864,.T.);
#49045=EDGE_CURVE('',#39328,#39329,#21321,.T.);
#49046=EDGE_CURVE('',#39329,#39330,#865,.T.);
#49047=EDGE_CURVE('',#39330,#39331,#21322,.T.);
#49048=EDGE_CURVE('',#39331,#39320,#21323,.T.);
#49049=EDGE_CURVE('',#39332,#39333,#866,.T.);
#49050=EDGE_CURVE('',#39333,#39334,#21324,.T.);
#49051=EDGE_CURVE('',#39334,#39335,#21325,.T.);
#49052=EDGE_CURVE('',#39335,#39336,#21326,.T.);
#49053=EDGE_CURVE('',#39336,#39337,#867,.T.);
#49054=EDGE_CURVE('',#39337,#39338,#21327,.T.);
#49055=EDGE_CURVE('',#39338,#39339,#21328,.T.);
#49056=EDGE_CURVE('',#39339,#39340,#868,.T.);
#49057=EDGE_CURVE('',#39340,#39341,#21329,.T.);
#49058=EDGE_CURVE('',#39341,#39342,#869,.T.);
#49059=EDGE_CURVE('',#39342,#39343,#21330,.T.);
#49060=EDGE_CURVE('',#39343,#39332,#21331,.T.);
#49061=EDGE_CURVE('',#39344,#39345,#21332,.T.);
#49062=EDGE_CURVE('',#39345,#39346,#31704,.T.);
#49063=EDGE_CURVE('',#39346,#39347,#21333,.T.);
#49064=EDGE_CURVE('',#39347,#39344,#31705,.T.);
#49065=EDGE_CURVE('',#39348,#39349,#870,.T.);
#49066=EDGE_CURVE('',#39349,#39350,#21334,.T.);
#49067=EDGE_CURVE('',#39350,#39351,#21335,.T.);
#49068=EDGE_CURVE('',#39351,#39352,#21336,.T.);
#49069=EDGE_CURVE('',#39352,#39353,#871,.T.);
#49070=EDGE_CURVE('',#39353,#39354,#21337,.T.);
#49071=EDGE_CURVE('',#39354,#39355,#21338,.T.);
#49072=EDGE_CURVE('',#39355,#39356,#872,.T.);
#49073=EDGE_CURVE('',#39356,#39357,#21339,.T.);
#49074=EDGE_CURVE('',#39357,#39358,#873,.T.);
#49075=EDGE_CURVE('',#39358,#39359,#21340,.T.);
#49076=EDGE_CURVE('',#39359,#39348,#21341,.T.);
#49077=EDGE_CURVE('',#39360,#39361,#874,.T.);
#49078=EDGE_CURVE('',#39361,#39362,#21342,.T.);
#49079=EDGE_CURVE('',#39362,#39363,#21343,.T.);
#49080=EDGE_CURVE('',#39363,#39364,#21344,.T.);
#49081=EDGE_CURVE('',#39364,#39365,#875,.T.);
#49082=EDGE_CURVE('',#39365,#39366,#21345,.T.);
#49083=EDGE_CURVE('',#39366,#39367,#21346,.T.);
#49084=EDGE_CURVE('',#39367,#39368,#876,.T.);
#49085=EDGE_CURVE('',#39368,#39369,#21347,.T.);
#49086=EDGE_CURVE('',#39369,#39370,#877,.T.);
#49087=EDGE_CURVE('',#39370,#39371,#21348,.T.);
#49088=EDGE_CURVE('',#39371,#39360,#21349,.T.);
#49089=EDGE_CURVE('',#39372,#39373,#21350,.T.);
#49090=EDGE_CURVE('',#39373,#39374,#31706,.T.);
#49091=EDGE_CURVE('',#39374,#39375,#21351,.T.);
#49092=EDGE_CURVE('',#39375,#39372,#31707,.T.);
#49093=EDGE_CURVE('',#39376,#39377,#878,.T.);
#49094=EDGE_CURVE('',#39377,#39378,#21352,.T.);
#49095=EDGE_CURVE('',#39378,#39379,#21353,.T.);
#49096=EDGE_CURVE('',#39379,#39380,#21354,.T.);
#49097=EDGE_CURVE('',#39380,#39381,#879,.T.);
#49098=EDGE_CURVE('',#39381,#39382,#21355,.T.);
#49099=EDGE_CURVE('',#39382,#39383,#21356,.T.);
#49100=EDGE_CURVE('',#39383,#39384,#880,.T.);
#49101=EDGE_CURVE('',#39384,#39385,#21357,.T.);
#49102=EDGE_CURVE('',#39385,#39386,#881,.T.);
#49103=EDGE_CURVE('',#39386,#39387,#21358,.T.);
#49104=EDGE_CURVE('',#39387,#39376,#21359,.T.);
#49105=EDGE_CURVE('',#39388,#39389,#882,.T.);
#49106=EDGE_CURVE('',#39389,#39390,#21360,.T.);
#49107=EDGE_CURVE('',#39390,#39391,#21361,.T.);
#49108=EDGE_CURVE('',#39391,#39392,#21362,.T.);
#49109=EDGE_CURVE('',#39392,#39393,#883,.T.);
#49110=EDGE_CURVE('',#39393,#39394,#21363,.T.);
#49111=EDGE_CURVE('',#39394,#39395,#21364,.T.);
#49112=EDGE_CURVE('',#39395,#39396,#884,.T.);
#49113=EDGE_CURVE('',#39396,#39397,#21365,.T.);
#49114=EDGE_CURVE('',#39397,#39398,#885,.T.);
#49115=EDGE_CURVE('',#39398,#39399,#21366,.T.);
#49116=EDGE_CURVE('',#39399,#39388,#21367,.T.);
#49117=EDGE_CURVE('',#39400,#39401,#21368,.T.);
#49118=EDGE_CURVE('',#39401,#39402,#31708,.T.);
#49119=EDGE_CURVE('',#39402,#39403,#21369,.T.);
#49120=EDGE_CURVE('',#39403,#39400,#31709,.T.);
#49121=EDGE_CURVE('',#39404,#39405,#886,.T.);
#49122=EDGE_CURVE('',#39405,#39406,#21370,.T.);
#49123=EDGE_CURVE('',#39406,#39407,#21371,.T.);
#49124=EDGE_CURVE('',#39407,#39408,#21372,.T.);
#49125=EDGE_CURVE('',#39408,#39409,#887,.T.);
#49126=EDGE_CURVE('',#39409,#39410,#21373,.T.);
#49127=EDGE_CURVE('',#39410,#39411,#21374,.T.);
#49128=EDGE_CURVE('',#39411,#39412,#888,.T.);
#49129=EDGE_CURVE('',#39412,#39413,#21375,.T.);
#49130=EDGE_CURVE('',#39413,#39414,#889,.T.);
#49131=EDGE_CURVE('',#39414,#39415,#21376,.T.);
#49132=EDGE_CURVE('',#39415,#39404,#21377,.T.);
#49133=EDGE_CURVE('',#39416,#39417,#890,.T.);
#49134=EDGE_CURVE('',#39417,#39418,#21378,.T.);
#49135=EDGE_CURVE('',#39418,#39419,#21379,.T.);
#49136=EDGE_CURVE('',#39419,#39420,#21380,.T.);
#49137=EDGE_CURVE('',#39420,#39421,#891,.T.);
#49138=EDGE_CURVE('',#39421,#39422,#21381,.T.);
#49139=EDGE_CURVE('',#39422,#39423,#21382,.T.);
#49140=EDGE_CURVE('',#39423,#39424,#892,.T.);
#49141=EDGE_CURVE('',#39424,#39425,#21383,.T.);
#49142=EDGE_CURVE('',#39425,#39426,#893,.T.);
#49143=EDGE_CURVE('',#39426,#39427,#21384,.T.);
#49144=EDGE_CURVE('',#39427,#39416,#21385,.T.);
#49145=EDGE_CURVE('',#39428,#39429,#21386,.T.);
#49146=EDGE_CURVE('',#39429,#39430,#31710,.T.);
#49147=EDGE_CURVE('',#39430,#39431,#21387,.T.);
#49148=EDGE_CURVE('',#39431,#39428,#31711,.T.);
#49149=EDGE_CURVE('',#39432,#39433,#894,.T.);
#49150=EDGE_CURVE('',#39433,#39434,#21388,.T.);
#49151=EDGE_CURVE('',#39434,#39435,#21389,.T.);
#49152=EDGE_CURVE('',#39435,#39436,#21390,.T.);
#49153=EDGE_CURVE('',#39436,#39437,#895,.T.);
#49154=EDGE_CURVE('',#39437,#39438,#21391,.T.);
#49155=EDGE_CURVE('',#39438,#39439,#21392,.T.);
#49156=EDGE_CURVE('',#39439,#39440,#896,.T.);
#49157=EDGE_CURVE('',#39440,#39441,#21393,.T.);
#49158=EDGE_CURVE('',#39441,#39442,#897,.T.);
#49159=EDGE_CURVE('',#39442,#39443,#21394,.T.);
#49160=EDGE_CURVE('',#39443,#39432,#21395,.T.);
#49161=EDGE_CURVE('',#39444,#39445,#898,.T.);
#49162=EDGE_CURVE('',#39445,#39446,#21396,.T.);
#49163=EDGE_CURVE('',#39446,#39447,#21397,.T.);
#49164=EDGE_CURVE('',#39447,#39448,#21398,.T.);
#49165=EDGE_CURVE('',#39448,#39449,#899,.T.);
#49166=EDGE_CURVE('',#39449,#39450,#21399,.T.);
#49167=EDGE_CURVE('',#39450,#39451,#21400,.T.);
#49168=EDGE_CURVE('',#39451,#39452,#900,.T.);
#49169=EDGE_CURVE('',#39452,#39453,#21401,.T.);
#49170=EDGE_CURVE('',#39453,#39454,#901,.T.);
#49171=EDGE_CURVE('',#39454,#39455,#21402,.T.);
#49172=EDGE_CURVE('',#39455,#39444,#21403,.T.);
#49173=EDGE_CURVE('',#39456,#39457,#21404,.T.);
#49174=EDGE_CURVE('',#39457,#39458,#31712,.T.);
#49175=EDGE_CURVE('',#39458,#39459,#21405,.T.);
#49176=EDGE_CURVE('',#39459,#39456,#31713,.T.);
#49177=EDGE_CURVE('',#39460,#39461,#902,.T.);
#49178=EDGE_CURVE('',#39461,#39462,#21406,.T.);
#49179=EDGE_CURVE('',#39462,#39463,#21407,.T.);
#49180=EDGE_CURVE('',#39463,#39464,#21408,.T.);
#49181=EDGE_CURVE('',#39464,#39465,#903,.T.);
#49182=EDGE_CURVE('',#39465,#39466,#21409,.T.);
#49183=EDGE_CURVE('',#39466,#39467,#21410,.T.);
#49184=EDGE_CURVE('',#39467,#39468,#904,.T.);
#49185=EDGE_CURVE('',#39468,#39469,#21411,.T.);
#49186=EDGE_CURVE('',#39469,#39470,#905,.T.);
#49187=EDGE_CURVE('',#39470,#39471,#21412,.T.);
#49188=EDGE_CURVE('',#39471,#39460,#21413,.T.);
#49189=EDGE_CURVE('',#39472,#39473,#906,.T.);
#49190=EDGE_CURVE('',#39473,#39474,#21414,.T.);
#49191=EDGE_CURVE('',#39474,#39475,#21415,.T.);
#49192=EDGE_CURVE('',#39475,#39476,#21416,.T.);
#49193=EDGE_CURVE('',#39476,#39477,#907,.T.);
#49194=EDGE_CURVE('',#39477,#39478,#21417,.T.);
#49195=EDGE_CURVE('',#39478,#39479,#21418,.T.);
#49196=EDGE_CURVE('',#39479,#39480,#908,.T.);
#49197=EDGE_CURVE('',#39480,#39481,#21419,.T.);
#49198=EDGE_CURVE('',#39481,#39482,#909,.T.);
#49199=EDGE_CURVE('',#39482,#39483,#21420,.T.);
#49200=EDGE_CURVE('',#39483,#39472,#21421,.T.);
#49201=EDGE_CURVE('',#39484,#39485,#21422,.T.);
#49202=EDGE_CURVE('',#39485,#39486,#31714,.T.);
#49203=EDGE_CURVE('',#39486,#39487,#21423,.T.);
#49204=EDGE_CURVE('',#39487,#39484,#31715,.T.);
#49205=EDGE_CURVE('',#39488,#39489,#910,.T.);
#49206=EDGE_CURVE('',#39489,#39490,#21424,.T.);
#49207=EDGE_CURVE('',#39490,#39491,#21425,.T.);
#49208=EDGE_CURVE('',#39491,#39492,#21426,.T.);
#49209=EDGE_CURVE('',#39492,#39493,#911,.T.);
#49210=EDGE_CURVE('',#39493,#39494,#21427,.T.);
#49211=EDGE_CURVE('',#39494,#39495,#21428,.T.);
#49212=EDGE_CURVE('',#39495,#39496,#912,.T.);
#49213=EDGE_CURVE('',#39496,#39497,#21429,.T.);
#49214=EDGE_CURVE('',#39497,#39498,#913,.T.);
#49215=EDGE_CURVE('',#39498,#39499,#21430,.T.);
#49216=EDGE_CURVE('',#39499,#39488,#21431,.T.);
#49217=EDGE_CURVE('',#39500,#39501,#914,.T.);
#49218=EDGE_CURVE('',#39501,#39502,#21432,.T.);
#49219=EDGE_CURVE('',#39502,#39503,#21433,.T.);
#49220=EDGE_CURVE('',#39503,#39504,#21434,.T.);
#49221=EDGE_CURVE('',#39504,#39505,#915,.T.);
#49222=EDGE_CURVE('',#39505,#39506,#21435,.T.);
#49223=EDGE_CURVE('',#39506,#39507,#21436,.T.);
#49224=EDGE_CURVE('',#39507,#39508,#916,.T.);
#49225=EDGE_CURVE('',#39508,#39509,#21437,.T.);
#49226=EDGE_CURVE('',#39509,#39510,#917,.T.);
#49227=EDGE_CURVE('',#39510,#39511,#21438,.T.);
#49228=EDGE_CURVE('',#39511,#39500,#21439,.T.);
#49229=EDGE_CURVE('',#39512,#39513,#21440,.T.);
#49230=EDGE_CURVE('',#39513,#39514,#31716,.T.);
#49231=EDGE_CURVE('',#39514,#39515,#21441,.T.);
#49232=EDGE_CURVE('',#39515,#39512,#31717,.T.);
#49233=EDGE_CURVE('',#39516,#39517,#918,.T.);
#49234=EDGE_CURVE('',#39517,#39518,#21442,.T.);
#49235=EDGE_CURVE('',#39518,#39519,#21443,.T.);
#49236=EDGE_CURVE('',#39519,#39520,#21444,.T.);
#49237=EDGE_CURVE('',#39520,#39521,#919,.T.);
#49238=EDGE_CURVE('',#39521,#39522,#21445,.T.);
#49239=EDGE_CURVE('',#39522,#39523,#21446,.T.);
#49240=EDGE_CURVE('',#39523,#39524,#920,.T.);
#49241=EDGE_CURVE('',#39524,#39525,#21447,.T.);
#49242=EDGE_CURVE('',#39525,#39526,#921,.T.);
#49243=EDGE_CURVE('',#39526,#39527,#21448,.T.);
#49244=EDGE_CURVE('',#39527,#39516,#21449,.T.);
#49245=EDGE_CURVE('',#39528,#39529,#922,.T.);
#49246=EDGE_CURVE('',#39529,#39530,#21450,.T.);
#49247=EDGE_CURVE('',#39530,#39531,#21451,.T.);
#49248=EDGE_CURVE('',#39531,#39532,#21452,.T.);
#49249=EDGE_CURVE('',#39532,#39533,#923,.T.);
#49250=EDGE_CURVE('',#39533,#39534,#21453,.T.);
#49251=EDGE_CURVE('',#39534,#39535,#21454,.T.);
#49252=EDGE_CURVE('',#39535,#39536,#924,.T.);
#49253=EDGE_CURVE('',#39536,#39537,#21455,.T.);
#49254=EDGE_CURVE('',#39537,#39538,#925,.T.);
#49255=EDGE_CURVE('',#39538,#39539,#21456,.T.);
#49256=EDGE_CURVE('',#39539,#39528,#21457,.T.);
#49257=EDGE_CURVE('',#39540,#39541,#21458,.T.);
#49258=EDGE_CURVE('',#39541,#39542,#31718,.T.);
#49259=EDGE_CURVE('',#39542,#39543,#21459,.T.);
#49260=EDGE_CURVE('',#39543,#39540,#31719,.T.);
#49261=EDGE_CURVE('',#39544,#39545,#926,.T.);
#49262=EDGE_CURVE('',#39545,#39546,#21460,.T.);
#49263=EDGE_CURVE('',#39546,#39547,#21461,.T.);
#49264=EDGE_CURVE('',#39547,#39548,#21462,.T.);
#49265=EDGE_CURVE('',#39548,#39549,#927,.T.);
#49266=EDGE_CURVE('',#39549,#39550,#21463,.T.);
#49267=EDGE_CURVE('',#39550,#39551,#21464,.T.);
#49268=EDGE_CURVE('',#39551,#39552,#928,.T.);
#49269=EDGE_CURVE('',#39552,#39553,#21465,.T.);
#49270=EDGE_CURVE('',#39553,#39554,#929,.T.);
#49271=EDGE_CURVE('',#39554,#39555,#21466,.T.);
#49272=EDGE_CURVE('',#39555,#39544,#21467,.T.);
#49273=EDGE_CURVE('',#39556,#39557,#930,.T.);
#49274=EDGE_CURVE('',#39557,#39558,#21468,.T.);
#49275=EDGE_CURVE('',#39558,#39559,#21469,.T.);
#49276=EDGE_CURVE('',#39559,#39560,#21470,.T.);
#49277=EDGE_CURVE('',#39560,#39561,#931,.T.);
#49278=EDGE_CURVE('',#39561,#39562,#21471,.T.);
#49279=EDGE_CURVE('',#39562,#39563,#21472,.T.);
#49280=EDGE_CURVE('',#39563,#39564,#932,.T.);
#49281=EDGE_CURVE('',#39564,#39565,#21473,.T.);
#49282=EDGE_CURVE('',#39565,#39566,#933,.T.);
#49283=EDGE_CURVE('',#39566,#39567,#21474,.T.);
#49284=EDGE_CURVE('',#39567,#39556,#21475,.T.);
#49285=EDGE_CURVE('',#39568,#39569,#21476,.T.);
#49286=EDGE_CURVE('',#39569,#39570,#31720,.T.);
#49287=EDGE_CURVE('',#39570,#39571,#21477,.T.);
#49288=EDGE_CURVE('',#39571,#39568,#31721,.T.);
#49289=EDGE_CURVE('',#39572,#39573,#934,.T.);
#49290=EDGE_CURVE('',#39573,#39574,#21478,.T.);
#49291=EDGE_CURVE('',#39574,#39575,#21479,.T.);
#49292=EDGE_CURVE('',#39575,#39576,#21480,.T.);
#49293=EDGE_CURVE('',#39576,#39577,#935,.T.);
#49294=EDGE_CURVE('',#39577,#39578,#21481,.T.);
#49295=EDGE_CURVE('',#39578,#39579,#21482,.T.);
#49296=EDGE_CURVE('',#39579,#39580,#936,.T.);
#49297=EDGE_CURVE('',#39580,#39581,#21483,.T.);
#49298=EDGE_CURVE('',#39581,#39582,#937,.T.);
#49299=EDGE_CURVE('',#39582,#39583,#21484,.T.);
#49300=EDGE_CURVE('',#39583,#39572,#21485,.T.);
#49301=EDGE_CURVE('',#39584,#39585,#938,.T.);
#49302=EDGE_CURVE('',#39585,#39586,#21486,.T.);
#49303=EDGE_CURVE('',#39586,#39587,#21487,.T.);
#49304=EDGE_CURVE('',#39587,#39588,#21488,.T.);
#49305=EDGE_CURVE('',#39588,#39589,#939,.T.);
#49306=EDGE_CURVE('',#39589,#39590,#21489,.T.);
#49307=EDGE_CURVE('',#39590,#39591,#21490,.T.);
#49308=EDGE_CURVE('',#39591,#39592,#940,.T.);
#49309=EDGE_CURVE('',#39592,#39593,#21491,.T.);
#49310=EDGE_CURVE('',#39593,#39594,#941,.T.);
#49311=EDGE_CURVE('',#39594,#39595,#21492,.T.);
#49312=EDGE_CURVE('',#39595,#39584,#21493,.T.);
#49313=EDGE_CURVE('',#36820,#36826,#21494,.T.);
#49314=EDGE_CURVE('',#36825,#36819,#21495,.T.);
#49315=EDGE_CURVE('',#39596,#39597,#942,.T.);
#49316=EDGE_CURVE('',#39597,#39598,#21496,.T.);
#49317=EDGE_CURVE('',#39598,#39599,#21497,.T.);
#49318=EDGE_CURVE('',#39599,#39600,#21498,.T.);
#49319=EDGE_CURVE('',#39600,#39601,#943,.T.);
#49320=EDGE_CURVE('',#39601,#39602,#21499,.T.);
#49321=EDGE_CURVE('',#39602,#39603,#21500,.T.);
#49322=EDGE_CURVE('',#39603,#39604,#944,.T.);
#49323=EDGE_CURVE('',#39604,#39605,#21501,.T.);
#49324=EDGE_CURVE('',#39605,#39606,#945,.T.);
#49325=EDGE_CURVE('',#39606,#39607,#21502,.T.);
#49326=EDGE_CURVE('',#39607,#39596,#21503,.T.);
#49327=EDGE_CURVE('',#39608,#39609,#946,.T.);
#49328=EDGE_CURVE('',#39609,#39610,#21504,.T.);
#49329=EDGE_CURVE('',#39610,#39611,#21505,.T.);
#49330=EDGE_CURVE('',#39611,#39612,#21506,.T.);
#49331=EDGE_CURVE('',#39612,#39613,#947,.T.);
#49332=EDGE_CURVE('',#39613,#39614,#21507,.T.);
#49333=EDGE_CURVE('',#39614,#39615,#21508,.T.);
#49334=EDGE_CURVE('',#39615,#39616,#948,.T.);
#49335=EDGE_CURVE('',#39616,#39617,#21509,.T.);
#49336=EDGE_CURVE('',#39617,#39618,#949,.T.);
#49337=EDGE_CURVE('',#39618,#39619,#21510,.T.);
#49338=EDGE_CURVE('',#39619,#39608,#21511,.T.);
#49339=EDGE_CURVE('',#39620,#39621,#21512,.T.);
#49340=EDGE_CURVE('',#39621,#39622,#31722,.T.);
#49341=EDGE_CURVE('',#39622,#39623,#21513,.T.);
#49342=EDGE_CURVE('',#39623,#39620,#31723,.T.);
#49343=EDGE_CURVE('',#39624,#39625,#950,.T.);
#49344=EDGE_CURVE('',#39625,#39626,#21514,.T.);
#49345=EDGE_CURVE('',#39626,#39627,#21515,.T.);
#49346=EDGE_CURVE('',#39627,#39628,#21516,.T.);
#49347=EDGE_CURVE('',#39628,#39629,#951,.T.);
#49348=EDGE_CURVE('',#39629,#39630,#21517,.T.);
#49349=EDGE_CURVE('',#39630,#39631,#21518,.T.);
#49350=EDGE_CURVE('',#39631,#39632,#952,.T.);
#49351=EDGE_CURVE('',#39632,#39633,#21519,.T.);
#49352=EDGE_CURVE('',#39633,#39634,#953,.T.);
#49353=EDGE_CURVE('',#39634,#39635,#21520,.T.);
#49354=EDGE_CURVE('',#39635,#39624,#21521,.T.);
#49355=EDGE_CURVE('',#39636,#39637,#954,.T.);
#49356=EDGE_CURVE('',#39637,#39638,#21522,.T.);
#49357=EDGE_CURVE('',#39638,#39639,#21523,.T.);
#49358=EDGE_CURVE('',#39639,#39640,#21524,.T.);
#49359=EDGE_CURVE('',#39640,#39641,#955,.T.);
#49360=EDGE_CURVE('',#39641,#39642,#21525,.T.);
#49361=EDGE_CURVE('',#39642,#39643,#21526,.T.);
#49362=EDGE_CURVE('',#39643,#39644,#956,.T.);
#49363=EDGE_CURVE('',#39644,#39645,#21527,.T.);
#49364=EDGE_CURVE('',#39645,#39646,#957,.T.);
#49365=EDGE_CURVE('',#39646,#39647,#21528,.T.);
#49366=EDGE_CURVE('',#39647,#39636,#21529,.T.);
#49367=EDGE_CURVE('',#39648,#39649,#21530,.T.);
#49368=EDGE_CURVE('',#39649,#39650,#31724,.T.);
#49369=EDGE_CURVE('',#39650,#39651,#21531,.T.);
#49370=EDGE_CURVE('',#39651,#39648,#31725,.T.);
#49371=EDGE_CURVE('',#39652,#39653,#958,.T.);
#49372=EDGE_CURVE('',#39653,#39654,#21532,.T.);
#49373=EDGE_CURVE('',#39654,#39655,#21533,.T.);
#49374=EDGE_CURVE('',#39655,#39656,#21534,.T.);
#49375=EDGE_CURVE('',#39656,#39657,#959,.T.);
#49376=EDGE_CURVE('',#39657,#39658,#21535,.T.);
#49377=EDGE_CURVE('',#39658,#39659,#21536,.T.);
#49378=EDGE_CURVE('',#39659,#39660,#960,.T.);
#49379=EDGE_CURVE('',#39660,#39661,#21537,.T.);
#49380=EDGE_CURVE('',#39661,#39662,#961,.T.);
#49381=EDGE_CURVE('',#39662,#39663,#21538,.T.);
#49382=EDGE_CURVE('',#39663,#39652,#21539,.T.);
#49383=EDGE_CURVE('',#39664,#39665,#962,.T.);
#49384=EDGE_CURVE('',#39665,#39666,#21540,.T.);
#49385=EDGE_CURVE('',#39666,#39667,#21541,.T.);
#49386=EDGE_CURVE('',#39667,#39668,#21542,.T.);
#49387=EDGE_CURVE('',#39668,#39669,#963,.T.);
#49388=EDGE_CURVE('',#39669,#39670,#21543,.T.);
#49389=EDGE_CURVE('',#39670,#39671,#21544,.T.);
#49390=EDGE_CURVE('',#39671,#39672,#964,.T.);
#49391=EDGE_CURVE('',#39672,#39673,#21545,.T.);
#49392=EDGE_CURVE('',#39673,#39674,#965,.T.);
#49393=EDGE_CURVE('',#39674,#39675,#21546,.T.);
#49394=EDGE_CURVE('',#39675,#39664,#21547,.T.);
#49395=EDGE_CURVE('',#39676,#39677,#21548,.T.);
#49396=EDGE_CURVE('',#39677,#39678,#31726,.T.);
#49397=EDGE_CURVE('',#39678,#39679,#21549,.T.);
#49398=EDGE_CURVE('',#39679,#39676,#31727,.T.);
#49399=EDGE_CURVE('',#39680,#39681,#966,.T.);
#49400=EDGE_CURVE('',#39681,#39682,#21550,.T.);
#49401=EDGE_CURVE('',#39682,#39683,#21551,.T.);
#49402=EDGE_CURVE('',#39683,#39684,#21552,.T.);
#49403=EDGE_CURVE('',#39684,#39685,#967,.T.);
#49404=EDGE_CURVE('',#39685,#39686,#21553,.T.);
#49405=EDGE_CURVE('',#39686,#39687,#21554,.T.);
#49406=EDGE_CURVE('',#39687,#39688,#968,.T.);
#49407=EDGE_CURVE('',#39688,#39689,#21555,.T.);
#49408=EDGE_CURVE('',#39689,#39690,#969,.T.);
#49409=EDGE_CURVE('',#39690,#39691,#21556,.T.);
#49410=EDGE_CURVE('',#39691,#39680,#21557,.T.);
#49411=EDGE_CURVE('',#39692,#39693,#970,.T.);
#49412=EDGE_CURVE('',#39693,#39694,#21558,.T.);
#49413=EDGE_CURVE('',#39694,#39695,#21559,.T.);
#49414=EDGE_CURVE('',#39695,#39696,#21560,.T.);
#49415=EDGE_CURVE('',#39696,#39697,#971,.T.);
#49416=EDGE_CURVE('',#39697,#39698,#21561,.T.);
#49417=EDGE_CURVE('',#39698,#39699,#21562,.T.);
#49418=EDGE_CURVE('',#39699,#39700,#972,.T.);
#49419=EDGE_CURVE('',#39700,#39701,#21563,.T.);
#49420=EDGE_CURVE('',#39701,#39702,#973,.T.);
#49421=EDGE_CURVE('',#39702,#39703,#21564,.T.);
#49422=EDGE_CURVE('',#39703,#39692,#21565,.T.);
#49423=EDGE_CURVE('',#39704,#39705,#21566,.T.);
#49424=EDGE_CURVE('',#39705,#39706,#31728,.T.);
#49425=EDGE_CURVE('',#39706,#39707,#21567,.T.);
#49426=EDGE_CURVE('',#39707,#39704,#31729,.T.);
#49427=EDGE_CURVE('',#39708,#39709,#974,.T.);
#49428=EDGE_CURVE('',#39709,#39710,#21568,.T.);
#49429=EDGE_CURVE('',#39710,#39711,#21569,.T.);
#49430=EDGE_CURVE('',#39711,#39712,#21570,.T.);
#49431=EDGE_CURVE('',#39712,#39713,#975,.T.);
#49432=EDGE_CURVE('',#39713,#39714,#21571,.T.);
#49433=EDGE_CURVE('',#39714,#39715,#21572,.T.);
#49434=EDGE_CURVE('',#39715,#39716,#976,.T.);
#49435=EDGE_CURVE('',#39716,#39717,#21573,.T.);
#49436=EDGE_CURVE('',#39717,#39718,#977,.T.);
#49437=EDGE_CURVE('',#39718,#39719,#21574,.T.);
#49438=EDGE_CURVE('',#39719,#39708,#21575,.T.);
#49439=EDGE_CURVE('',#39720,#39721,#978,.T.);
#49440=EDGE_CURVE('',#39721,#39722,#21576,.T.);
#49441=EDGE_CURVE('',#39722,#39723,#21577,.T.);
#49442=EDGE_CURVE('',#39723,#39724,#21578,.T.);
#49443=EDGE_CURVE('',#39724,#39725,#979,.T.);
#49444=EDGE_CURVE('',#39725,#39726,#21579,.T.);
#49445=EDGE_CURVE('',#39726,#39727,#21580,.T.);
#49446=EDGE_CURVE('',#39727,#39728,#980,.T.);
#49447=EDGE_CURVE('',#39728,#39729,#21581,.T.);
#49448=EDGE_CURVE('',#39729,#39730,#981,.T.);
#49449=EDGE_CURVE('',#39730,#39731,#21582,.T.);
#49450=EDGE_CURVE('',#39731,#39720,#21583,.T.);
#49451=EDGE_CURVE('',#39732,#39733,#21584,.T.);
#49452=EDGE_CURVE('',#39733,#39734,#31730,.T.);
#49453=EDGE_CURVE('',#39734,#39735,#21585,.T.);
#49454=EDGE_CURVE('',#39735,#39732,#31731,.T.);
#49455=EDGE_CURVE('',#39736,#39737,#982,.T.);
#49456=EDGE_CURVE('',#39737,#39738,#21586,.T.);
#49457=EDGE_CURVE('',#39738,#39739,#21587,.T.);
#49458=EDGE_CURVE('',#39739,#39740,#21588,.T.);
#49459=EDGE_CURVE('',#39740,#39741,#983,.T.);
#49460=EDGE_CURVE('',#39741,#39742,#21589,.T.);
#49461=EDGE_CURVE('',#39742,#39743,#21590,.T.);
#49462=EDGE_CURVE('',#39743,#39744,#984,.T.);
#49463=EDGE_CURVE('',#39744,#39745,#21591,.T.);
#49464=EDGE_CURVE('',#39745,#39746,#985,.T.);
#49465=EDGE_CURVE('',#39746,#39747,#21592,.T.);
#49466=EDGE_CURVE('',#39747,#39736,#21593,.T.);
#49467=EDGE_CURVE('',#39748,#39749,#986,.T.);
#49468=EDGE_CURVE('',#39749,#39750,#21594,.T.);
#49469=EDGE_CURVE('',#39750,#39751,#21595,.T.);
#49470=EDGE_CURVE('',#39751,#39752,#21596,.T.);
#49471=EDGE_CURVE('',#39752,#39753,#987,.T.);
#49472=EDGE_CURVE('',#39753,#39754,#21597,.T.);
#49473=EDGE_CURVE('',#39754,#39755,#21598,.T.);
#49474=EDGE_CURVE('',#39755,#39756,#988,.T.);
#49475=EDGE_CURVE('',#39756,#39757,#21599,.T.);
#49476=EDGE_CURVE('',#39757,#39758,#989,.T.);
#49477=EDGE_CURVE('',#39758,#39759,#21600,.T.);
#49478=EDGE_CURVE('',#39759,#39748,#21601,.T.);
#49479=EDGE_CURVE('',#39760,#39761,#21602,.T.);
#49480=EDGE_CURVE('',#39761,#39762,#31732,.T.);
#49481=EDGE_CURVE('',#39762,#39763,#21603,.T.);
#49482=EDGE_CURVE('',#39763,#39760,#31733,.T.);
#49483=EDGE_CURVE('',#39764,#39765,#990,.T.);
#49484=EDGE_CURVE('',#39765,#39766,#21604,.T.);
#49485=EDGE_CURVE('',#39766,#39767,#21605,.T.);
#49486=EDGE_CURVE('',#39767,#39768,#21606,.T.);
#49487=EDGE_CURVE('',#39768,#39769,#991,.T.);
#49488=EDGE_CURVE('',#39769,#39770,#21607,.T.);
#49489=EDGE_CURVE('',#39770,#39771,#21608,.T.);
#49490=EDGE_CURVE('',#39771,#39772,#992,.T.);
#49491=EDGE_CURVE('',#39772,#39773,#21609,.T.);
#49492=EDGE_CURVE('',#39773,#39774,#993,.T.);
#49493=EDGE_CURVE('',#39774,#39775,#21610,.T.);
#49494=EDGE_CURVE('',#39775,#39764,#21611,.T.);
#49495=EDGE_CURVE('',#39776,#39777,#994,.T.);
#49496=EDGE_CURVE('',#39777,#39778,#21612,.T.);
#49497=EDGE_CURVE('',#39778,#39779,#21613,.T.);
#49498=EDGE_CURVE('',#39779,#39780,#21614,.T.);
#49499=EDGE_CURVE('',#39780,#39781,#995,.T.);
#49500=EDGE_CURVE('',#39781,#39782,#21615,.T.);
#49501=EDGE_CURVE('',#39782,#39783,#21616,.T.);
#49502=EDGE_CURVE('',#39783,#39784,#996,.T.);
#49503=EDGE_CURVE('',#39784,#39785,#21617,.T.);
#49504=EDGE_CURVE('',#39785,#39786,#997,.T.);
#49505=EDGE_CURVE('',#39786,#39787,#21618,.T.);
#49506=EDGE_CURVE('',#39787,#39776,#21619,.T.);
#49507=EDGE_CURVE('',#39788,#39789,#21620,.T.);
#49508=EDGE_CURVE('',#39789,#39790,#31734,.T.);
#49509=EDGE_CURVE('',#39790,#39791,#21621,.T.);
#49510=EDGE_CURVE('',#39791,#39788,#31735,.T.);
#49511=EDGE_CURVE('',#39792,#39793,#998,.T.);
#49512=EDGE_CURVE('',#39793,#39794,#21622,.T.);
#49513=EDGE_CURVE('',#39794,#39795,#21623,.T.);
#49514=EDGE_CURVE('',#39795,#39796,#21624,.T.);
#49515=EDGE_CURVE('',#39796,#39797,#999,.T.);
#49516=EDGE_CURVE('',#39797,#39798,#21625,.T.);
#49517=EDGE_CURVE('',#39798,#39799,#21626,.T.);
#49518=EDGE_CURVE('',#39799,#39800,#1000,.T.);
#49519=EDGE_CURVE('',#39800,#39801,#21627,.T.);
#49520=EDGE_CURVE('',#39801,#39802,#1001,.T.);
#49521=EDGE_CURVE('',#39802,#39803,#21628,.T.);
#49522=EDGE_CURVE('',#39803,#39792,#21629,.T.);
#49523=EDGE_CURVE('',#39804,#39805,#1002,.T.);
#49524=EDGE_CURVE('',#39805,#39806,#21630,.T.);
#49525=EDGE_CURVE('',#39806,#39807,#21631,.T.);
#49526=EDGE_CURVE('',#39807,#39808,#21632,.T.);
#49527=EDGE_CURVE('',#39808,#39809,#1003,.T.);
#49528=EDGE_CURVE('',#39809,#39810,#21633,.T.);
#49529=EDGE_CURVE('',#39810,#39811,#21634,.T.);
#49530=EDGE_CURVE('',#39811,#39812,#1004,.T.);
#49531=EDGE_CURVE('',#39812,#39813,#21635,.T.);
#49532=EDGE_CURVE('',#39813,#39814,#1005,.T.);
#49533=EDGE_CURVE('',#39814,#39815,#21636,.T.);
#49534=EDGE_CURVE('',#39815,#39804,#21637,.T.);
#49535=EDGE_CURVE('',#39816,#39817,#21638,.T.);
#49536=EDGE_CURVE('',#39817,#39818,#31736,.T.);
#49537=EDGE_CURVE('',#39818,#39819,#21639,.T.);
#49538=EDGE_CURVE('',#39819,#39816,#31737,.T.);
#49539=EDGE_CURVE('',#39820,#39821,#1006,.T.);
#49540=EDGE_CURVE('',#39821,#39822,#21640,.T.);
#49541=EDGE_CURVE('',#39822,#39823,#21641,.T.);
#49542=EDGE_CURVE('',#39823,#39824,#21642,.T.);
#49543=EDGE_CURVE('',#39824,#39825,#1007,.T.);
#49544=EDGE_CURVE('',#39825,#39826,#21643,.T.);
#49545=EDGE_CURVE('',#39826,#39827,#21644,.T.);
#49546=EDGE_CURVE('',#39827,#39828,#1008,.T.);
#49547=EDGE_CURVE('',#39828,#39829,#21645,.T.);
#49548=EDGE_CURVE('',#39829,#39830,#1009,.T.);
#49549=EDGE_CURVE('',#39830,#39831,#21646,.T.);
#49550=EDGE_CURVE('',#39831,#39820,#21647,.T.);
#49551=EDGE_CURVE('',#39832,#39833,#1010,.T.);
#49552=EDGE_CURVE('',#39833,#39834,#21648,.T.);
#49553=EDGE_CURVE('',#39834,#39835,#21649,.T.);
#49554=EDGE_CURVE('',#39835,#39836,#21650,.T.);
#49555=EDGE_CURVE('',#39836,#39837,#1011,.T.);
#49556=EDGE_CURVE('',#39837,#39838,#21651,.T.);
#49557=EDGE_CURVE('',#39838,#39839,#21652,.T.);
#49558=EDGE_CURVE('',#39839,#39840,#1012,.T.);
#49559=EDGE_CURVE('',#39840,#39841,#21653,.T.);
#49560=EDGE_CURVE('',#39841,#39842,#1013,.T.);
#49561=EDGE_CURVE('',#39842,#39843,#21654,.T.);
#49562=EDGE_CURVE('',#39843,#39832,#21655,.T.);
#49563=EDGE_CURVE('',#39844,#39845,#21656,.T.);
#49564=EDGE_CURVE('',#39845,#39846,#31738,.T.);
#49565=EDGE_CURVE('',#39846,#39847,#21657,.T.);
#49566=EDGE_CURVE('',#39847,#39844,#31739,.T.);
#49567=EDGE_CURVE('',#39848,#39849,#1014,.T.);
#49568=EDGE_CURVE('',#39849,#39850,#21658,.T.);
#49569=EDGE_CURVE('',#39850,#39851,#21659,.T.);
#49570=EDGE_CURVE('',#39851,#39852,#21660,.T.);
#49571=EDGE_CURVE('',#39852,#39853,#1015,.T.);
#49572=EDGE_CURVE('',#39853,#39854,#21661,.T.);
#49573=EDGE_CURVE('',#39854,#39855,#21662,.T.);
#49574=EDGE_CURVE('',#39855,#39856,#1016,.T.);
#49575=EDGE_CURVE('',#39856,#39857,#21663,.T.);
#49576=EDGE_CURVE('',#39857,#39858,#1017,.T.);
#49577=EDGE_CURVE('',#39858,#39859,#21664,.T.);
#49578=EDGE_CURVE('',#39859,#39848,#21665,.T.);
#49579=EDGE_CURVE('',#39860,#39861,#1018,.T.);
#49580=EDGE_CURVE('',#39861,#39862,#21666,.T.);
#49581=EDGE_CURVE('',#39862,#39863,#21667,.T.);
#49582=EDGE_CURVE('',#39863,#39864,#21668,.T.);
#49583=EDGE_CURVE('',#39864,#39865,#1019,.T.);
#49584=EDGE_CURVE('',#39865,#39866,#21669,.T.);
#49585=EDGE_CURVE('',#39866,#39867,#21670,.T.);
#49586=EDGE_CURVE('',#39867,#39868,#1020,.T.);
#49587=EDGE_CURVE('',#39868,#39869,#21671,.T.);
#49588=EDGE_CURVE('',#39869,#39870,#1021,.T.);
#49589=EDGE_CURVE('',#39870,#39871,#21672,.T.);
#49590=EDGE_CURVE('',#39871,#39860,#21673,.T.);
#49591=EDGE_CURVE('',#39872,#39873,#21674,.T.);
#49592=EDGE_CURVE('',#39873,#39874,#31740,.T.);
#49593=EDGE_CURVE('',#39874,#39875,#21675,.T.);
#49594=EDGE_CURVE('',#39875,#39872,#31741,.T.);
#49595=EDGE_CURVE('',#39876,#39877,#1022,.T.);
#49596=EDGE_CURVE('',#39877,#39878,#21676,.T.);
#49597=EDGE_CURVE('',#39878,#39879,#21677,.T.);
#49598=EDGE_CURVE('',#39879,#39880,#21678,.T.);
#49599=EDGE_CURVE('',#39880,#39881,#1023,.T.);
#49600=EDGE_CURVE('',#39881,#39882,#21679,.T.);
#49601=EDGE_CURVE('',#39882,#39883,#21680,.T.);
#49602=EDGE_CURVE('',#39883,#39884,#1024,.T.);
#49603=EDGE_CURVE('',#39884,#39885,#21681,.T.);
#49604=EDGE_CURVE('',#39885,#39886,#1025,.T.);
#49605=EDGE_CURVE('',#39886,#39887,#21682,.T.);
#49606=EDGE_CURVE('',#39887,#39876,#21683,.T.);
#49607=EDGE_CURVE('',#39888,#39889,#1026,.T.);
#49608=EDGE_CURVE('',#39889,#39890,#21684,.T.);
#49609=EDGE_CURVE('',#39890,#39891,#21685,.T.);
#49610=EDGE_CURVE('',#39891,#39892,#21686,.T.);
#49611=EDGE_CURVE('',#39892,#39893,#1027,.T.);
#49612=EDGE_CURVE('',#39893,#39894,#21687,.T.);
#49613=EDGE_CURVE('',#39894,#39895,#21688,.T.);
#49614=EDGE_CURVE('',#39895,#39896,#1028,.T.);
#49615=EDGE_CURVE('',#39896,#39897,#21689,.T.);
#49616=EDGE_CURVE('',#39897,#39898,#1029,.T.);
#49617=EDGE_CURVE('',#39898,#39899,#21690,.T.);
#49618=EDGE_CURVE('',#39899,#39888,#21691,.T.);
#49619=EDGE_CURVE('',#39900,#39901,#21692,.T.);
#49620=EDGE_CURVE('',#39901,#39902,#31742,.T.);
#49621=EDGE_CURVE('',#39902,#39903,#21693,.T.);
#49622=EDGE_CURVE('',#39903,#39900,#31743,.T.);
#49623=EDGE_CURVE('',#39904,#39905,#1030,.T.);
#49624=EDGE_CURVE('',#39905,#39906,#21694,.T.);
#49625=EDGE_CURVE('',#39906,#39907,#21695,.T.);
#49626=EDGE_CURVE('',#39907,#39908,#21696,.T.);
#49627=EDGE_CURVE('',#39908,#39909,#1031,.T.);
#49628=EDGE_CURVE('',#39909,#39910,#21697,.T.);
#49629=EDGE_CURVE('',#39910,#39911,#21698,.T.);
#49630=EDGE_CURVE('',#39911,#39912,#1032,.T.);
#49631=EDGE_CURVE('',#39912,#39913,#21699,.T.);
#49632=EDGE_CURVE('',#39913,#39914,#1033,.T.);
#49633=EDGE_CURVE('',#39914,#39915,#21700,.T.);
#49634=EDGE_CURVE('',#39915,#39904,#21701,.T.);
#49635=EDGE_CURVE('',#39916,#39917,#1034,.T.);
#49636=EDGE_CURVE('',#39917,#39918,#21702,.T.);
#49637=EDGE_CURVE('',#39918,#39919,#21703,.T.);
#49638=EDGE_CURVE('',#39919,#39920,#21704,.T.);
#49639=EDGE_CURVE('',#39920,#39921,#1035,.T.);
#49640=EDGE_CURVE('',#39921,#39922,#21705,.T.);
#49641=EDGE_CURVE('',#39922,#39923,#21706,.T.);
#49642=EDGE_CURVE('',#39923,#39924,#1036,.T.);
#49643=EDGE_CURVE('',#39924,#39925,#21707,.T.);
#49644=EDGE_CURVE('',#39925,#39926,#1037,.T.);
#49645=EDGE_CURVE('',#39926,#39927,#21708,.T.);
#49646=EDGE_CURVE('',#39927,#39916,#21709,.T.);
#49647=EDGE_CURVE('',#39928,#39929,#21710,.T.);
#49648=EDGE_CURVE('',#39929,#39930,#31744,.T.);
#49649=EDGE_CURVE('',#39930,#39931,#21711,.T.);
#49650=EDGE_CURVE('',#39931,#39928,#31745,.T.);
#49651=EDGE_CURVE('',#39932,#39933,#1038,.T.);
#49652=EDGE_CURVE('',#39933,#39934,#21712,.T.);
#49653=EDGE_CURVE('',#39934,#39935,#21713,.T.);
#49654=EDGE_CURVE('',#39935,#39936,#21714,.T.);
#49655=EDGE_CURVE('',#39936,#39937,#1039,.T.);
#49656=EDGE_CURVE('',#39937,#39938,#21715,.T.);
#49657=EDGE_CURVE('',#39938,#39939,#21716,.T.);
#49658=EDGE_CURVE('',#39939,#39940,#1040,.T.);
#49659=EDGE_CURVE('',#39940,#39941,#21717,.T.);
#49660=EDGE_CURVE('',#39941,#39942,#1041,.T.);
#49661=EDGE_CURVE('',#39942,#39943,#21718,.T.);
#49662=EDGE_CURVE('',#39943,#39932,#21719,.T.);
#49663=EDGE_CURVE('',#39944,#39945,#1042,.T.);
#49664=EDGE_CURVE('',#39945,#39946,#21720,.T.);
#49665=EDGE_CURVE('',#39946,#39947,#21721,.T.);
#49666=EDGE_CURVE('',#39947,#39948,#21722,.T.);
#49667=EDGE_CURVE('',#39948,#39949,#1043,.T.);
#49668=EDGE_CURVE('',#39949,#39950,#21723,.T.);
#49669=EDGE_CURVE('',#39950,#39951,#21724,.T.);
#49670=EDGE_CURVE('',#39951,#39952,#1044,.T.);
#49671=EDGE_CURVE('',#39952,#39953,#21725,.T.);
#49672=EDGE_CURVE('',#39953,#39954,#1045,.T.);
#49673=EDGE_CURVE('',#39954,#39955,#21726,.T.);
#49674=EDGE_CURVE('',#39955,#39944,#21727,.T.);
#49675=EDGE_CURVE('',#39956,#39957,#21728,.T.);
#49676=EDGE_CURVE('',#39957,#39958,#31746,.T.);
#49677=EDGE_CURVE('',#39958,#39959,#21729,.T.);
#49678=EDGE_CURVE('',#39959,#39956,#31747,.T.);
#49679=EDGE_CURVE('',#39960,#39961,#1046,.T.);
#49680=EDGE_CURVE('',#39961,#39962,#21730,.T.);
#49681=EDGE_CURVE('',#39962,#39963,#21731,.T.);
#49682=EDGE_CURVE('',#39963,#39964,#21732,.T.);
#49683=EDGE_CURVE('',#39964,#39965,#1047,.T.);
#49684=EDGE_CURVE('',#39965,#39966,#21733,.T.);
#49685=EDGE_CURVE('',#39966,#39967,#21734,.T.);
#49686=EDGE_CURVE('',#39967,#39968,#1048,.T.);
#49687=EDGE_CURVE('',#39968,#39969,#21735,.T.);
#49688=EDGE_CURVE('',#39969,#39970,#1049,.T.);
#49689=EDGE_CURVE('',#39970,#39971,#21736,.T.);
#49690=EDGE_CURVE('',#39971,#39960,#21737,.T.);
#49691=EDGE_CURVE('',#39972,#39973,#1050,.T.);
#49692=EDGE_CURVE('',#39973,#39974,#21738,.T.);
#49693=EDGE_CURVE('',#39974,#39975,#21739,.T.);
#49694=EDGE_CURVE('',#39975,#39976,#21740,.T.);
#49695=EDGE_CURVE('',#39976,#39977,#1051,.T.);
#49696=EDGE_CURVE('',#39977,#39978,#21741,.T.);
#49697=EDGE_CURVE('',#39978,#39979,#21742,.T.);
#49698=EDGE_CURVE('',#39979,#39980,#1052,.T.);
#49699=EDGE_CURVE('',#39980,#39981,#21743,.T.);
#49700=EDGE_CURVE('',#39981,#39982,#1053,.T.);
#49701=EDGE_CURVE('',#39982,#39983,#21744,.T.);
#49702=EDGE_CURVE('',#39983,#39972,#21745,.T.);
#49703=EDGE_CURVE('',#39984,#39985,#21746,.T.);
#49704=EDGE_CURVE('',#39985,#39986,#31748,.T.);
#49705=EDGE_CURVE('',#39986,#39987,#21747,.T.);
#49706=EDGE_CURVE('',#39987,#39984,#31749,.T.);
#49707=EDGE_CURVE('',#39988,#39989,#1054,.T.);
#49708=EDGE_CURVE('',#39989,#39990,#21748,.T.);
#49709=EDGE_CURVE('',#39990,#39991,#21749,.T.);
#49710=EDGE_CURVE('',#39991,#39992,#21750,.T.);
#49711=EDGE_CURVE('',#39992,#39993,#1055,.T.);
#49712=EDGE_CURVE('',#39993,#39994,#21751,.T.);
#49713=EDGE_CURVE('',#39994,#39995,#21752,.T.);
#49714=EDGE_CURVE('',#39995,#39996,#1056,.T.);
#49715=EDGE_CURVE('',#39996,#39997,#21753,.T.);
#49716=EDGE_CURVE('',#39997,#39998,#1057,.T.);
#49717=EDGE_CURVE('',#39998,#39999,#21754,.T.);
#49718=EDGE_CURVE('',#39999,#39988,#21755,.T.);
#49719=EDGE_CURVE('',#40000,#40001,#1058,.T.);
#49720=EDGE_CURVE('',#40001,#40002,#21756,.T.);
#49721=EDGE_CURVE('',#40002,#40003,#21757,.T.);
#49722=EDGE_CURVE('',#40003,#40004,#21758,.T.);
#49723=EDGE_CURVE('',#40004,#40005,#1059,.T.);
#49724=EDGE_CURVE('',#40005,#40006,#21759,.T.);
#49725=EDGE_CURVE('',#40006,#40007,#21760,.T.);
#49726=EDGE_CURVE('',#40007,#40008,#1060,.T.);
#49727=EDGE_CURVE('',#40008,#40009,#21761,.T.);
#49728=EDGE_CURVE('',#40009,#40010,#1061,.T.);
#49729=EDGE_CURVE('',#40010,#40011,#21762,.T.);
#49730=EDGE_CURVE('',#40011,#40000,#21763,.T.);
#49731=EDGE_CURVE('',#36812,#36818,#21764,.T.);
#49732=EDGE_CURVE('',#36817,#36811,#21765,.T.);
#49733=EDGE_CURVE('',#40012,#40013,#1062,.T.);
#49734=EDGE_CURVE('',#40013,#40014,#21766,.T.);
#49735=EDGE_CURVE('',#40014,#40015,#21767,.T.);
#49736=EDGE_CURVE('',#40015,#40016,#21768,.T.);
#49737=EDGE_CURVE('',#40016,#40017,#1063,.T.);
#49738=EDGE_CURVE('',#40017,#40018,#21769,.T.);
#49739=EDGE_CURVE('',#40018,#40019,#21770,.T.);
#49740=EDGE_CURVE('',#40019,#40020,#1064,.T.);
#49741=EDGE_CURVE('',#40020,#40021,#21771,.T.);
#49742=EDGE_CURVE('',#40021,#40022,#1065,.T.);
#49743=EDGE_CURVE('',#40022,#40023,#21772,.T.);
#49744=EDGE_CURVE('',#40023,#40012,#21773,.T.);
#49745=EDGE_CURVE('',#40024,#40025,#1066,.T.);
#49746=EDGE_CURVE('',#40025,#40026,#21774,.T.);
#49747=EDGE_CURVE('',#40026,#40027,#21775,.T.);
#49748=EDGE_CURVE('',#40027,#40028,#21776,.T.);
#49749=EDGE_CURVE('',#40028,#40029,#1067,.T.);
#49750=EDGE_CURVE('',#40029,#40030,#21777,.T.);
#49751=EDGE_CURVE('',#40030,#40031,#21778,.T.);
#49752=EDGE_CURVE('',#40031,#40032,#1068,.T.);
#49753=EDGE_CURVE('',#40032,#40033,#21779,.T.);
#49754=EDGE_CURVE('',#40033,#40034,#1069,.T.);
#49755=EDGE_CURVE('',#40034,#40035,#21780,.T.);
#49756=EDGE_CURVE('',#40035,#40024,#21781,.T.);
#49757=EDGE_CURVE('',#40036,#40037,#21782,.T.);
#49758=EDGE_CURVE('',#40037,#40038,#31750,.T.);
#49759=EDGE_CURVE('',#40038,#40039,#21783,.T.);
#49760=EDGE_CURVE('',#40039,#40036,#31751,.T.);
#49761=EDGE_CURVE('',#40040,#40041,#1070,.T.);
#49762=EDGE_CURVE('',#40041,#40042,#21784,.T.);
#49763=EDGE_CURVE('',#40042,#40043,#21785,.T.);
#49764=EDGE_CURVE('',#40043,#40044,#21786,.T.);
#49765=EDGE_CURVE('',#40044,#40045,#1071,.T.);
#49766=EDGE_CURVE('',#40045,#40046,#21787,.T.);
#49767=EDGE_CURVE('',#40046,#40047,#21788,.T.);
#49768=EDGE_CURVE('',#40047,#40048,#1072,.T.);
#49769=EDGE_CURVE('',#40048,#40049,#21789,.T.);
#49770=EDGE_CURVE('',#40049,#40050,#1073,.T.);
#49771=EDGE_CURVE('',#40050,#40051,#21790,.T.);
#49772=EDGE_CURVE('',#40051,#40040,#21791,.T.);
#49773=EDGE_CURVE('',#40052,#40053,#1074,.T.);
#49774=EDGE_CURVE('',#40053,#40054,#21792,.T.);
#49775=EDGE_CURVE('',#40054,#40055,#21793,.T.);
#49776=EDGE_CURVE('',#40055,#40056,#21794,.T.);
#49777=EDGE_CURVE('',#40056,#40057,#1075,.T.);
#49778=EDGE_CURVE('',#40057,#40058,#21795,.T.);
#49779=EDGE_CURVE('',#40058,#40059,#21796,.T.);
#49780=EDGE_CURVE('',#40059,#40060,#1076,.T.);
#49781=EDGE_CURVE('',#40060,#40061,#21797,.T.);
#49782=EDGE_CURVE('',#40061,#40062,#1077,.T.);
#49783=EDGE_CURVE('',#40062,#40063,#21798,.T.);
#49784=EDGE_CURVE('',#40063,#40052,#21799,.T.);
#49785=EDGE_CURVE('',#40064,#40065,#21800,.T.);
#49786=EDGE_CURVE('',#40065,#40066,#31752,.T.);
#49787=EDGE_CURVE('',#40066,#40067,#21801,.T.);
#49788=EDGE_CURVE('',#40067,#40064,#31753,.T.);
#49789=EDGE_CURVE('',#40068,#40069,#1078,.T.);
#49790=EDGE_CURVE('',#40069,#40070,#21802,.T.);
#49791=EDGE_CURVE('',#40070,#40071,#21803,.T.);
#49792=EDGE_CURVE('',#40071,#40072,#21804,.T.);
#49793=EDGE_CURVE('',#40072,#40073,#1079,.T.);
#49794=EDGE_CURVE('',#40073,#40074,#21805,.T.);
#49795=EDGE_CURVE('',#40074,#40075,#21806,.T.);
#49796=EDGE_CURVE('',#40075,#40076,#1080,.T.);
#49797=EDGE_CURVE('',#40076,#40077,#21807,.T.);
#49798=EDGE_CURVE('',#40077,#40078,#1081,.T.);
#49799=EDGE_CURVE('',#40078,#40079,#21808,.T.);
#49800=EDGE_CURVE('',#40079,#40068,#21809,.T.);
#49801=EDGE_CURVE('',#40080,#40081,#1082,.T.);
#49802=EDGE_CURVE('',#40081,#40082,#21810,.T.);
#49803=EDGE_CURVE('',#40082,#40083,#21811,.T.);
#49804=EDGE_CURVE('',#40083,#40084,#21812,.T.);
#49805=EDGE_CURVE('',#40084,#40085,#1083,.T.);
#49806=EDGE_CURVE('',#40085,#40086,#21813,.T.);
#49807=EDGE_CURVE('',#40086,#40087,#21814,.T.);
#49808=EDGE_CURVE('',#40087,#40088,#1084,.T.);
#49809=EDGE_CURVE('',#40088,#40089,#21815,.T.);
#49810=EDGE_CURVE('',#40089,#40090,#1085,.T.);
#49811=EDGE_CURVE('',#40090,#40091,#21816,.T.);
#49812=EDGE_CURVE('',#40091,#40080,#21817,.T.);
#49813=EDGE_CURVE('',#40092,#40093,#21818,.T.);
#49814=EDGE_CURVE('',#40093,#40094,#31754,.T.);
#49815=EDGE_CURVE('',#40094,#40095,#21819,.T.);
#49816=EDGE_CURVE('',#40095,#40092,#31755,.T.);
#49817=EDGE_CURVE('',#40096,#40097,#1086,.T.);
#49818=EDGE_CURVE('',#40097,#40098,#21820,.T.);
#49819=EDGE_CURVE('',#40098,#40099,#21821,.T.);
#49820=EDGE_CURVE('',#40099,#40100,#21822,.T.);
#49821=EDGE_CURVE('',#40100,#40101,#1087,.T.);
#49822=EDGE_CURVE('',#40101,#40102,#21823,.T.);
#49823=EDGE_CURVE('',#40102,#40103,#21824,.T.);
#49824=EDGE_CURVE('',#40103,#40104,#1088,.T.);
#49825=EDGE_CURVE('',#40104,#40105,#21825,.T.);
#49826=EDGE_CURVE('',#40105,#40106,#1089,.T.);
#49827=EDGE_CURVE('',#40106,#40107,#21826,.T.);
#49828=EDGE_CURVE('',#40107,#40096,#21827,.T.);
#49829=EDGE_CURVE('',#40108,#40109,#1090,.T.);
#49830=EDGE_CURVE('',#40109,#40110,#21828,.T.);
#49831=EDGE_CURVE('',#40110,#40111,#21829,.T.);
#49832=EDGE_CURVE('',#40111,#40112,#21830,.T.);
#49833=EDGE_CURVE('',#40112,#40113,#1091,.T.);
#49834=EDGE_CURVE('',#40113,#40114,#21831,.T.);
#49835=EDGE_CURVE('',#40114,#40115,#21832,.T.);
#49836=EDGE_CURVE('',#40115,#40116,#1092,.T.);
#49837=EDGE_CURVE('',#40116,#40117,#21833,.T.);
#49838=EDGE_CURVE('',#40117,#40118,#1093,.T.);
#49839=EDGE_CURVE('',#40118,#40119,#21834,.T.);
#49840=EDGE_CURVE('',#40119,#40108,#21835,.T.);
#49841=EDGE_CURVE('',#40120,#40121,#21836,.T.);
#49842=EDGE_CURVE('',#40121,#40122,#31756,.T.);
#49843=EDGE_CURVE('',#40122,#40123,#21837,.T.);
#49844=EDGE_CURVE('',#40123,#40120,#31757,.T.);
#49845=EDGE_CURVE('',#40124,#40125,#1094,.T.);
#49846=EDGE_CURVE('',#40125,#40126,#21838,.T.);
#49847=EDGE_CURVE('',#40126,#40127,#21839,.T.);
#49848=EDGE_CURVE('',#40127,#40128,#21840,.T.);
#49849=EDGE_CURVE('',#40128,#40129,#1095,.T.);
#49850=EDGE_CURVE('',#40129,#40130,#21841,.T.);
#49851=EDGE_CURVE('',#40130,#40131,#21842,.T.);
#49852=EDGE_CURVE('',#40131,#40132,#1096,.T.);
#49853=EDGE_CURVE('',#40132,#40133,#21843,.T.);
#49854=EDGE_CURVE('',#40133,#40134,#1097,.T.);
#49855=EDGE_CURVE('',#40134,#40135,#21844,.T.);
#49856=EDGE_CURVE('',#40135,#40124,#21845,.T.);
#49857=EDGE_CURVE('',#40136,#40137,#1098,.T.);
#49858=EDGE_CURVE('',#40137,#40138,#21846,.T.);
#49859=EDGE_CURVE('',#40138,#40139,#21847,.T.);
#49860=EDGE_CURVE('',#40139,#40140,#21848,.T.);
#49861=EDGE_CURVE('',#40140,#40141,#1099,.T.);
#49862=EDGE_CURVE('',#40141,#40142,#21849,.T.);
#49863=EDGE_CURVE('',#40142,#40143,#21850,.T.);
#49864=EDGE_CURVE('',#40143,#40144,#1100,.T.);
#49865=EDGE_CURVE('',#40144,#40145,#21851,.T.);
#49866=EDGE_CURVE('',#40145,#40146,#1101,.T.);
#49867=EDGE_CURVE('',#40146,#40147,#21852,.T.);
#49868=EDGE_CURVE('',#40147,#40136,#21853,.T.);
#49869=EDGE_CURVE('',#40148,#40149,#21854,.T.);
#49870=EDGE_CURVE('',#40149,#40150,#31758,.T.);
#49871=EDGE_CURVE('',#40150,#40151,#21855,.T.);
#49872=EDGE_CURVE('',#40151,#40148,#31759,.T.);
#49873=EDGE_CURVE('',#40152,#40153,#1102,.T.);
#49874=EDGE_CURVE('',#40153,#40154,#21856,.T.);
#49875=EDGE_CURVE('',#40154,#40155,#21857,.T.);
#49876=EDGE_CURVE('',#40155,#40156,#21858,.T.);
#49877=EDGE_CURVE('',#40156,#40157,#1103,.T.);
#49878=EDGE_CURVE('',#40157,#40158,#21859,.T.);
#49879=EDGE_CURVE('',#40158,#40159,#21860,.T.);
#49880=EDGE_CURVE('',#40159,#40160,#1104,.T.);
#49881=EDGE_CURVE('',#40160,#40161,#21861,.T.);
#49882=EDGE_CURVE('',#40161,#40162,#1105,.T.);
#49883=EDGE_CURVE('',#40162,#40163,#21862,.T.);
#49884=EDGE_CURVE('',#40163,#40152,#21863,.T.);
#49885=EDGE_CURVE('',#40164,#40165,#1106,.T.);
#49886=EDGE_CURVE('',#40165,#40166,#21864,.T.);
#49887=EDGE_CURVE('',#40166,#40167,#21865,.T.);
#49888=EDGE_CURVE('',#40167,#40168,#21866,.T.);
#49889=EDGE_CURVE('',#40168,#40169,#1107,.T.);
#49890=EDGE_CURVE('',#40169,#40170,#21867,.T.);
#49891=EDGE_CURVE('',#40170,#40171,#21868,.T.);
#49892=EDGE_CURVE('',#40171,#40172,#1108,.T.);
#49893=EDGE_CURVE('',#40172,#40173,#21869,.T.);
#49894=EDGE_CURVE('',#40173,#40174,#1109,.T.);
#49895=EDGE_CURVE('',#40174,#40175,#21870,.T.);
#49896=EDGE_CURVE('',#40175,#40164,#21871,.T.);
#49897=EDGE_CURVE('',#40176,#40177,#21872,.T.);
#49898=EDGE_CURVE('',#40177,#40178,#31760,.T.);
#49899=EDGE_CURVE('',#40178,#40179,#21873,.T.);
#49900=EDGE_CURVE('',#40179,#40176,#31761,.T.);
#49901=EDGE_CURVE('',#40180,#40181,#1110,.T.);
#49902=EDGE_CURVE('',#40181,#40182,#21874,.T.);
#49903=EDGE_CURVE('',#40182,#40183,#21875,.T.);
#49904=EDGE_CURVE('',#40183,#40184,#21876,.T.);
#49905=EDGE_CURVE('',#40184,#40185,#1111,.T.);
#49906=EDGE_CURVE('',#40185,#40186,#21877,.T.);
#49907=EDGE_CURVE('',#40186,#40187,#21878,.T.);
#49908=EDGE_CURVE('',#40187,#40188,#1112,.T.);
#49909=EDGE_CURVE('',#40188,#40189,#21879,.T.);
#49910=EDGE_CURVE('',#40189,#40190,#1113,.T.);
#49911=EDGE_CURVE('',#40190,#40191,#21880,.T.);
#49912=EDGE_CURVE('',#40191,#40180,#21881,.T.);
#49913=EDGE_CURVE('',#40192,#40193,#1114,.T.);
#49914=EDGE_CURVE('',#40193,#40194,#21882,.T.);
#49915=EDGE_CURVE('',#40194,#40195,#21883,.T.);
#49916=EDGE_CURVE('',#40195,#40196,#21884,.T.);
#49917=EDGE_CURVE('',#40196,#40197,#1115,.T.);
#49918=EDGE_CURVE('',#40197,#40198,#21885,.T.);
#49919=EDGE_CURVE('',#40198,#40199,#21886,.T.);
#49920=EDGE_CURVE('',#40199,#40200,#1116,.T.);
#49921=EDGE_CURVE('',#40200,#40201,#21887,.T.);
#49922=EDGE_CURVE('',#40201,#40202,#1117,.T.);
#49923=EDGE_CURVE('',#40202,#40203,#21888,.T.);
#49924=EDGE_CURVE('',#40203,#40192,#21889,.T.);
#49925=EDGE_CURVE('',#40204,#40205,#21890,.T.);
#49926=EDGE_CURVE('',#40205,#40206,#31762,.T.);
#49927=EDGE_CURVE('',#40206,#40207,#21891,.T.);
#49928=EDGE_CURVE('',#40207,#40204,#31763,.T.);
#49929=EDGE_CURVE('',#40208,#40209,#1118,.T.);
#49930=EDGE_CURVE('',#40209,#40210,#21892,.T.);
#49931=EDGE_CURVE('',#40210,#40211,#21893,.T.);
#49932=EDGE_CURVE('',#40211,#40212,#21894,.T.);
#49933=EDGE_CURVE('',#40212,#40213,#1119,.T.);
#49934=EDGE_CURVE('',#40213,#40214,#21895,.T.);
#49935=EDGE_CURVE('',#40214,#40215,#21896,.T.);
#49936=EDGE_CURVE('',#40215,#40216,#1120,.T.);
#49937=EDGE_CURVE('',#40216,#40217,#21897,.T.);
#49938=EDGE_CURVE('',#40217,#40218,#1121,.T.);
#49939=EDGE_CURVE('',#40218,#40219,#21898,.T.);
#49940=EDGE_CURVE('',#40219,#40208,#21899,.T.);
#49941=EDGE_CURVE('',#40220,#40221,#1122,.T.);
#49942=EDGE_CURVE('',#40221,#40222,#21900,.T.);
#49943=EDGE_CURVE('',#40222,#40223,#21901,.T.);
#49944=EDGE_CURVE('',#40223,#40224,#21902,.T.);
#49945=EDGE_CURVE('',#40224,#40225,#1123,.T.);
#49946=EDGE_CURVE('',#40225,#40226,#21903,.T.);
#49947=EDGE_CURVE('',#40226,#40227,#21904,.T.);
#49948=EDGE_CURVE('',#40227,#40228,#1124,.T.);
#49949=EDGE_CURVE('',#40228,#40229,#21905,.T.);
#49950=EDGE_CURVE('',#40229,#40230,#1125,.T.);
#49951=EDGE_CURVE('',#40230,#40231,#21906,.T.);
#49952=EDGE_CURVE('',#40231,#40220,#21907,.T.);
#49953=EDGE_CURVE('',#40232,#40233,#21908,.T.);
#49954=EDGE_CURVE('',#40233,#40234,#31764,.T.);
#49955=EDGE_CURVE('',#40234,#40235,#21909,.T.);
#49956=EDGE_CURVE('',#40235,#40232,#31765,.T.);
#49957=EDGE_CURVE('',#40236,#40237,#1126,.T.);
#49958=EDGE_CURVE('',#40237,#40238,#21910,.T.);
#49959=EDGE_CURVE('',#40238,#40239,#21911,.T.);
#49960=EDGE_CURVE('',#40239,#40240,#21912,.T.);
#49961=EDGE_CURVE('',#40240,#40241,#1127,.T.);
#49962=EDGE_CURVE('',#40241,#40242,#21913,.T.);
#49963=EDGE_CURVE('',#40242,#40243,#21914,.T.);
#49964=EDGE_CURVE('',#40243,#40244,#1128,.T.);
#49965=EDGE_CURVE('',#40244,#40245,#21915,.T.);
#49966=EDGE_CURVE('',#40245,#40246,#1129,.T.);
#49967=EDGE_CURVE('',#40246,#40247,#21916,.T.);
#49968=EDGE_CURVE('',#40247,#40236,#21917,.T.);
#49969=EDGE_CURVE('',#40248,#40249,#1130,.T.);
#49970=EDGE_CURVE('',#40249,#40250,#21918,.T.);
#49971=EDGE_CURVE('',#40250,#40251,#21919,.T.);
#49972=EDGE_CURVE('',#40251,#40252,#21920,.T.);
#49973=EDGE_CURVE('',#40252,#40253,#1131,.T.);
#49974=EDGE_CURVE('',#40253,#40254,#21921,.T.);
#49975=EDGE_CURVE('',#40254,#40255,#21922,.T.);
#49976=EDGE_CURVE('',#40255,#40256,#1132,.T.);
#49977=EDGE_CURVE('',#40256,#40257,#21923,.T.);
#49978=EDGE_CURVE('',#40257,#40258,#1133,.T.);
#49979=EDGE_CURVE('',#40258,#40259,#21924,.T.);
#49980=EDGE_CURVE('',#40259,#40248,#21925,.T.);
#49981=EDGE_CURVE('',#40260,#40261,#21926,.T.);
#49982=EDGE_CURVE('',#40261,#40262,#31766,.T.);
#49983=EDGE_CURVE('',#40262,#40263,#21927,.T.);
#49984=EDGE_CURVE('',#40263,#40260,#31767,.T.);
#49985=EDGE_CURVE('',#40264,#40265,#1134,.T.);
#49986=EDGE_CURVE('',#40265,#40266,#21928,.T.);
#49987=EDGE_CURVE('',#40266,#40267,#21929,.T.);
#49988=EDGE_CURVE('',#40267,#40268,#21930,.T.);
#49989=EDGE_CURVE('',#40268,#40269,#1135,.T.);
#49990=EDGE_CURVE('',#40269,#40270,#21931,.T.);
#49991=EDGE_CURVE('',#40270,#40271,#21932,.T.);
#49992=EDGE_CURVE('',#40271,#40272,#1136,.T.);
#49993=EDGE_CURVE('',#40272,#40273,#21933,.T.);
#49994=EDGE_CURVE('',#40273,#40274,#1137,.T.);
#49995=EDGE_CURVE('',#40274,#40275,#21934,.T.);
#49996=EDGE_CURVE('',#40275,#40264,#21935,.T.);
#49997=EDGE_CURVE('',#40276,#40277,#1138,.T.);
#49998=EDGE_CURVE('',#40277,#40278,#21936,.T.);
#49999=EDGE_CURVE('',#40278,#40279,#21937,.T.);
#50000=EDGE_CURVE('',#40279,#40280,#21938,.T.);
#50001=EDGE_CURVE('',#40280,#40281,#1139,.T.);
#50002=EDGE_CURVE('',#40281,#40282,#21939,.T.);
#50003=EDGE_CURVE('',#40282,#40283,#21940,.T.);
#50004=EDGE_CURVE('',#40283,#40284,#1140,.T.);
#50005=EDGE_CURVE('',#40284,#40285,#21941,.T.);
#50006=EDGE_CURVE('',#40285,#40286,#1141,.T.);
#50007=EDGE_CURVE('',#40286,#40287,#21942,.T.);
#50008=EDGE_CURVE('',#40287,#40276,#21943,.T.);
#50009=EDGE_CURVE('',#40288,#40289,#21944,.T.);
#50010=EDGE_CURVE('',#40289,#40290,#31768,.T.);
#50011=EDGE_CURVE('',#40290,#40291,#21945,.T.);
#50012=EDGE_CURVE('',#40291,#40288,#31769,.T.);
#50013=EDGE_CURVE('',#40292,#40293,#1142,.T.);
#50014=EDGE_CURVE('',#40293,#40294,#21946,.T.);
#50015=EDGE_CURVE('',#40294,#40295,#21947,.T.);
#50016=EDGE_CURVE('',#40295,#40296,#21948,.T.);
#50017=EDGE_CURVE('',#40296,#40297,#1143,.T.);
#50018=EDGE_CURVE('',#40297,#40298,#21949,.T.);
#50019=EDGE_CURVE('',#40298,#40299,#21950,.T.);
#50020=EDGE_CURVE('',#40299,#40300,#1144,.T.);
#50021=EDGE_CURVE('',#40300,#40301,#21951,.T.);
#50022=EDGE_CURVE('',#40301,#40302,#1145,.T.);
#50023=EDGE_CURVE('',#40302,#40303,#21952,.T.);
#50024=EDGE_CURVE('',#40303,#40292,#21953,.T.);
#50025=EDGE_CURVE('',#40304,#40305,#1146,.T.);
#50026=EDGE_CURVE('',#40305,#40306,#21954,.T.);
#50027=EDGE_CURVE('',#40306,#40307,#21955,.T.);
#50028=EDGE_CURVE('',#40307,#40308,#21956,.T.);
#50029=EDGE_CURVE('',#40308,#40309,#1147,.T.);
#50030=EDGE_CURVE('',#40309,#40310,#21957,.T.);
#50031=EDGE_CURVE('',#40310,#40311,#21958,.T.);
#50032=EDGE_CURVE('',#40311,#40312,#1148,.T.);
#50033=EDGE_CURVE('',#40312,#40313,#21959,.T.);
#50034=EDGE_CURVE('',#40313,#40314,#1149,.T.);
#50035=EDGE_CURVE('',#40314,#40315,#21960,.T.);
#50036=EDGE_CURVE('',#40315,#40304,#21961,.T.);
#50037=EDGE_CURVE('',#40316,#40317,#21962,.T.);
#50038=EDGE_CURVE('',#40317,#40318,#31770,.T.);
#50039=EDGE_CURVE('',#40318,#40319,#21963,.T.);
#50040=EDGE_CURVE('',#40319,#40316,#31771,.T.);
#50041=EDGE_CURVE('',#40320,#40321,#1150,.T.);
#50042=EDGE_CURVE('',#40321,#40322,#21964,.T.);
#50043=EDGE_CURVE('',#40322,#40323,#21965,.T.);
#50044=EDGE_CURVE('',#40323,#40324,#21966,.T.);
#50045=EDGE_CURVE('',#40324,#40325,#1151,.T.);
#50046=EDGE_CURVE('',#40325,#40326,#21967,.T.);
#50047=EDGE_CURVE('',#40326,#40327,#21968,.T.);
#50048=EDGE_CURVE('',#40327,#40328,#1152,.T.);
#50049=EDGE_CURVE('',#40328,#40329,#21969,.T.);
#50050=EDGE_CURVE('',#40329,#40330,#1153,.T.);
#50051=EDGE_CURVE('',#40330,#40331,#21970,.T.);
#50052=EDGE_CURVE('',#40331,#40320,#21971,.T.);
#50053=EDGE_CURVE('',#40332,#40333,#1154,.T.);
#50054=EDGE_CURVE('',#40333,#40334,#21972,.T.);
#50055=EDGE_CURVE('',#40334,#40335,#21973,.T.);
#50056=EDGE_CURVE('',#40335,#40336,#21974,.T.);
#50057=EDGE_CURVE('',#40336,#40337,#1155,.T.);
#50058=EDGE_CURVE('',#40337,#40338,#21975,.T.);
#50059=EDGE_CURVE('',#40338,#40339,#21976,.T.);
#50060=EDGE_CURVE('',#40339,#40340,#1156,.T.);
#50061=EDGE_CURVE('',#40340,#40341,#21977,.T.);
#50062=EDGE_CURVE('',#40341,#40342,#1157,.T.);
#50063=EDGE_CURVE('',#40342,#40343,#21978,.T.);
#50064=EDGE_CURVE('',#40343,#40332,#21979,.T.);
#50065=EDGE_CURVE('',#40344,#40345,#21980,.T.);
#50066=EDGE_CURVE('',#40345,#40346,#31772,.T.);
#50067=EDGE_CURVE('',#40346,#40347,#21981,.T.);
#50068=EDGE_CURVE('',#40347,#40344,#31773,.T.);
#50069=EDGE_CURVE('',#40348,#40349,#1158,.T.);
#50070=EDGE_CURVE('',#40349,#40350,#21982,.T.);
#50071=EDGE_CURVE('',#40350,#40351,#21983,.T.);
#50072=EDGE_CURVE('',#40351,#40352,#21984,.T.);
#50073=EDGE_CURVE('',#40352,#40353,#1159,.T.);
#50074=EDGE_CURVE('',#40353,#40354,#21985,.T.);
#50075=EDGE_CURVE('',#40354,#40355,#21986,.T.);
#50076=EDGE_CURVE('',#40355,#40356,#1160,.T.);
#50077=EDGE_CURVE('',#40356,#40357,#21987,.T.);
#50078=EDGE_CURVE('',#40357,#40358,#1161,.T.);
#50079=EDGE_CURVE('',#40358,#40359,#21988,.T.);
#50080=EDGE_CURVE('',#40359,#40348,#21989,.T.);
#50081=EDGE_CURVE('',#40360,#40361,#1162,.T.);
#50082=EDGE_CURVE('',#40361,#40362,#21990,.T.);
#50083=EDGE_CURVE('',#40362,#40363,#21991,.T.);
#50084=EDGE_CURVE('',#40363,#40364,#21992,.T.);
#50085=EDGE_CURVE('',#40364,#40365,#1163,.T.);
#50086=EDGE_CURVE('',#40365,#40366,#21993,.T.);
#50087=EDGE_CURVE('',#40366,#40367,#21994,.T.);
#50088=EDGE_CURVE('',#40367,#40368,#1164,.T.);
#50089=EDGE_CURVE('',#40368,#40369,#21995,.T.);
#50090=EDGE_CURVE('',#40369,#40370,#1165,.T.);
#50091=EDGE_CURVE('',#40370,#40371,#21996,.T.);
#50092=EDGE_CURVE('',#40371,#40360,#21997,.T.);
#50093=EDGE_CURVE('',#40372,#40373,#21998,.T.);
#50094=EDGE_CURVE('',#40373,#40374,#31774,.T.);
#50095=EDGE_CURVE('',#40374,#40375,#21999,.T.);
#50096=EDGE_CURVE('',#40375,#40372,#31775,.T.);
#50097=EDGE_CURVE('',#40376,#40377,#1166,.T.);
#50098=EDGE_CURVE('',#40377,#40378,#22000,.T.);
#50099=EDGE_CURVE('',#40378,#40379,#22001,.T.);
#50100=EDGE_CURVE('',#40379,#40380,#22002,.T.);
#50101=EDGE_CURVE('',#40380,#40381,#1167,.T.);
#50102=EDGE_CURVE('',#40381,#40382,#22003,.T.);
#50103=EDGE_CURVE('',#40382,#40383,#22004,.T.);
#50104=EDGE_CURVE('',#40383,#40384,#1168,.T.);
#50105=EDGE_CURVE('',#40384,#40385,#22005,.T.);
#50106=EDGE_CURVE('',#40385,#40386,#1169,.T.);
#50107=EDGE_CURVE('',#40386,#40387,#22006,.T.);
#50108=EDGE_CURVE('',#40387,#40376,#22007,.T.);
#50109=EDGE_CURVE('',#40388,#40389,#1170,.T.);
#50110=EDGE_CURVE('',#40389,#40390,#22008,.T.);
#50111=EDGE_CURVE('',#40390,#40391,#22009,.T.);
#50112=EDGE_CURVE('',#40391,#40392,#22010,.T.);
#50113=EDGE_CURVE('',#40392,#40393,#1171,.T.);
#50114=EDGE_CURVE('',#40393,#40394,#22011,.T.);
#50115=EDGE_CURVE('',#40394,#40395,#22012,.T.);
#50116=EDGE_CURVE('',#40395,#40396,#1172,.T.);
#50117=EDGE_CURVE('',#40396,#40397,#22013,.T.);
#50118=EDGE_CURVE('',#40397,#40398,#1173,.T.);
#50119=EDGE_CURVE('',#40398,#40399,#22014,.T.);
#50120=EDGE_CURVE('',#40399,#40388,#22015,.T.);
#50121=EDGE_CURVE('',#40400,#40401,#22016,.T.);
#50122=EDGE_CURVE('',#40401,#40402,#31776,.T.);
#50123=EDGE_CURVE('',#40402,#40403,#22017,.T.);
#50124=EDGE_CURVE('',#40403,#40400,#31777,.T.);
#50125=EDGE_CURVE('',#40404,#40405,#1174,.T.);
#50126=EDGE_CURVE('',#40405,#40406,#22018,.T.);
#50127=EDGE_CURVE('',#40406,#40407,#22019,.T.);
#50128=EDGE_CURVE('',#40407,#40408,#22020,.T.);
#50129=EDGE_CURVE('',#40408,#40409,#1175,.T.);
#50130=EDGE_CURVE('',#40409,#40410,#22021,.T.);
#50131=EDGE_CURVE('',#40410,#40411,#22022,.T.);
#50132=EDGE_CURVE('',#40411,#40412,#1176,.T.);
#50133=EDGE_CURVE('',#40412,#40413,#22023,.T.);
#50134=EDGE_CURVE('',#40413,#40414,#1177,.T.);
#50135=EDGE_CURVE('',#40414,#40415,#22024,.T.);
#50136=EDGE_CURVE('',#40415,#40404,#22025,.T.);
#50137=EDGE_CURVE('',#40416,#40417,#1178,.T.);
#50138=EDGE_CURVE('',#40417,#40418,#22026,.T.);
#50139=EDGE_CURVE('',#40418,#40419,#22027,.T.);
#50140=EDGE_CURVE('',#40419,#40420,#22028,.T.);
#50141=EDGE_CURVE('',#40420,#40421,#1179,.T.);
#50142=EDGE_CURVE('',#40421,#40422,#22029,.T.);
#50143=EDGE_CURVE('',#40422,#40423,#22030,.T.);
#50144=EDGE_CURVE('',#40423,#40424,#1180,.T.);
#50145=EDGE_CURVE('',#40424,#40425,#22031,.T.);
#50146=EDGE_CURVE('',#40425,#40426,#1181,.T.);
#50147=EDGE_CURVE('',#40426,#40427,#22032,.T.);
#50148=EDGE_CURVE('',#40427,#40416,#22033,.T.);
#50149=EDGE_CURVE('',#38802,#38785,#4499,.T.);
#50150=EDGE_CURVE('',#38784,#38803,#4500,.T.);
#50151=EDGE_CURVE('',#38786,#38791,#4501,.T.);
#50152=EDGE_CURVE('',#38790,#38787,#4502,.T.);
#50153=EDGE_CURVE('',#38830,#38813,#4503,.T.);
#50154=EDGE_CURVE('',#38812,#38831,#4504,.T.);
#50155=EDGE_CURVE('',#38814,#38819,#4505,.T.);
#50156=EDGE_CURVE('',#38818,#38815,#4506,.T.);
#50157=EDGE_CURVE('',#38858,#38841,#4507,.T.);
#50158=EDGE_CURVE('',#38840,#38859,#4508,.T.);
#50159=EDGE_CURVE('',#38842,#38847,#4509,.T.);
#50160=EDGE_CURVE('',#38846,#38843,#4510,.T.);
#50161=EDGE_CURVE('',#38886,#38869,#4511,.T.);
#50162=EDGE_CURVE('',#38868,#38887,#4512,.T.);
#50163=EDGE_CURVE('',#38870,#38875,#4513,.T.);
#50164=EDGE_CURVE('',#38874,#38871,#4514,.T.);
#50165=EDGE_CURVE('',#38914,#38897,#4515,.T.);
#50166=EDGE_CURVE('',#38896,#38915,#4516,.T.);
#50167=EDGE_CURVE('',#38898,#38903,#4517,.T.);
#50168=EDGE_CURVE('',#38902,#38899,#4518,.T.);
#50169=EDGE_CURVE('',#38942,#38925,#4519,.T.);
#50170=EDGE_CURVE('',#38924,#38943,#4520,.T.);
#50171=EDGE_CURVE('',#38926,#38931,#4521,.T.);
#50172=EDGE_CURVE('',#38930,#38927,#4522,.T.);
#50173=EDGE_CURVE('',#38970,#38953,#4523,.T.);
#50174=EDGE_CURVE('',#38952,#38971,#4524,.T.);
#50175=EDGE_CURVE('',#38954,#38959,#4525,.T.);
#50176=EDGE_CURVE('',#38958,#38955,#4526,.T.);
#50177=EDGE_CURVE('',#38998,#38981,#4527,.T.);
#50178=EDGE_CURVE('',#38980,#38999,#4528,.T.);
#50179=EDGE_CURVE('',#38982,#38987,#4529,.T.);
#50180=EDGE_CURVE('',#38986,#38983,#4530,.T.);
#50181=EDGE_CURVE('',#39026,#39009,#4531,.T.);
#50182=EDGE_CURVE('',#39008,#39027,#4532,.T.);
#50183=EDGE_CURVE('',#39010,#39015,#4533,.T.);
#50184=EDGE_CURVE('',#39014,#39011,#4534,.T.);
#50185=EDGE_CURVE('',#39054,#39037,#4535,.T.);
#50186=EDGE_CURVE('',#39036,#39055,#4536,.T.);
#50187=EDGE_CURVE('',#39038,#39043,#4537,.T.);
#50188=EDGE_CURVE('',#39042,#39039,#4538,.T.);
#50189=EDGE_CURVE('',#39082,#39065,#4539,.T.);
#50190=EDGE_CURVE('',#39064,#39083,#4540,.T.);
#50191=EDGE_CURVE('',#39066,#39071,#4541,.T.);
#50192=EDGE_CURVE('',#39070,#39067,#4542,.T.);
#50193=EDGE_CURVE('',#39110,#39093,#4543,.T.);
#50194=EDGE_CURVE('',#39092,#39111,#4544,.T.);
#50195=EDGE_CURVE('',#39094,#39099,#4545,.T.);
#50196=EDGE_CURVE('',#39098,#39095,#4546,.T.);
#50197=EDGE_CURVE('',#39138,#39121,#4547,.T.);
#50198=EDGE_CURVE('',#39120,#39139,#4548,.T.);
#50199=EDGE_CURVE('',#39122,#39127,#4549,.T.);
#50200=EDGE_CURVE('',#39126,#39123,#4550,.T.);
#50201=EDGE_CURVE('',#39166,#39149,#4551,.T.);
#50202=EDGE_CURVE('',#39148,#39167,#4552,.T.);
#50203=EDGE_CURVE('',#39150,#39155,#4553,.T.);
#50204=EDGE_CURVE('',#39154,#39151,#4554,.T.);
#50205=EDGE_CURVE('',#39194,#39177,#4555,.T.);
#50206=EDGE_CURVE('',#39176,#39195,#4556,.T.);
#50207=EDGE_CURVE('',#39178,#39183,#4557,.T.);
#50208=EDGE_CURVE('',#39182,#39179,#4558,.T.);
#50209=EDGE_CURVE('',#39222,#39205,#4559,.T.);
#50210=EDGE_CURVE('',#39204,#39223,#4560,.T.);
#50211=EDGE_CURVE('',#39206,#39211,#4561,.T.);
#50212=EDGE_CURVE('',#39210,#39207,#4562,.T.);
#50213=EDGE_CURVE('',#39250,#39233,#4563,.T.);
#50214=EDGE_CURVE('',#39232,#39251,#4564,.T.);
#50215=EDGE_CURVE('',#39234,#39239,#4565,.T.);
#50216=EDGE_CURVE('',#39238,#39235,#4566,.T.);
#50217=EDGE_CURVE('',#39278,#39261,#4567,.T.);
#50218=EDGE_CURVE('',#39260,#39279,#4568,.T.);
#50219=EDGE_CURVE('',#39262,#39267,#4569,.T.);
#50220=EDGE_CURVE('',#39266,#39263,#4570,.T.);
#50221=EDGE_CURVE('',#39306,#39289,#4571,.T.);
#50222=EDGE_CURVE('',#39288,#39307,#4572,.T.);
#50223=EDGE_CURVE('',#39290,#39295,#4573,.T.);
#50224=EDGE_CURVE('',#39294,#39291,#4574,.T.);
#50225=EDGE_CURVE('',#39334,#39317,#4575,.T.);
#50226=EDGE_CURVE('',#39316,#39335,#4576,.T.);
#50227=EDGE_CURVE('',#39318,#39323,#4577,.T.);
#50228=EDGE_CURVE('',#39322,#39319,#4578,.T.);
#50229=EDGE_CURVE('',#39362,#39345,#4579,.T.);
#50230=EDGE_CURVE('',#39344,#39363,#4580,.T.);
#50231=EDGE_CURVE('',#39346,#39351,#4581,.T.);
#50232=EDGE_CURVE('',#39350,#39347,#4582,.T.);
#50233=EDGE_CURVE('',#39390,#39373,#4583,.T.);
#50234=EDGE_CURVE('',#39372,#39391,#4584,.T.);
#50235=EDGE_CURVE('',#39374,#39379,#4585,.T.);
#50236=EDGE_CURVE('',#39378,#39375,#4586,.T.);
#50237=EDGE_CURVE('',#39418,#39401,#4587,.T.);
#50238=EDGE_CURVE('',#39400,#39419,#4588,.T.);
#50239=EDGE_CURVE('',#39402,#39407,#4589,.T.);
#50240=EDGE_CURVE('',#39406,#39403,#4590,.T.);
#50241=EDGE_CURVE('',#39446,#39429,#4591,.T.);
#50242=EDGE_CURVE('',#39428,#39447,#4592,.T.);
#50243=EDGE_CURVE('',#39430,#39435,#4593,.T.);
#50244=EDGE_CURVE('',#39434,#39431,#4594,.T.);
#50245=EDGE_CURVE('',#39474,#39457,#4595,.T.);
#50246=EDGE_CURVE('',#39456,#39475,#4596,.T.);
#50247=EDGE_CURVE('',#39458,#39463,#4597,.T.);
#50248=EDGE_CURVE('',#39462,#39459,#4598,.T.);
#50249=EDGE_CURVE('',#39502,#39485,#4599,.T.);
#50250=EDGE_CURVE('',#39484,#39503,#4600,.T.);
#50251=EDGE_CURVE('',#39486,#39491,#4601,.T.);
#50252=EDGE_CURVE('',#39490,#39487,#4602,.T.);
#50253=EDGE_CURVE('',#39530,#39513,#4603,.T.);
#50254=EDGE_CURVE('',#39512,#39531,#4604,.T.);
#50255=EDGE_CURVE('',#39514,#39519,#4605,.T.);
#50256=EDGE_CURVE('',#39518,#39515,#4606,.T.);
#50257=EDGE_CURVE('',#39558,#39541,#4607,.T.);
#50258=EDGE_CURVE('',#39540,#39559,#4608,.T.);
#50259=EDGE_CURVE('',#39542,#39547,#4609,.T.);
#50260=EDGE_CURVE('',#39546,#39543,#4610,.T.);
#50261=EDGE_CURVE('',#39586,#39569,#4611,.T.);
#50262=EDGE_CURVE('',#39568,#39587,#4612,.T.);
#50263=EDGE_CURVE('',#39570,#39575,#4613,.T.);
#50264=EDGE_CURVE('',#39574,#39571,#4614,.T.);
#50265=EDGE_CURVE('',#39610,#36826,#4615,.T.);
#50266=EDGE_CURVE('',#36820,#39611,#4616,.T.);
#50267=EDGE_CURVE('',#36825,#39599,#4617,.T.);
#50268=EDGE_CURVE('',#39598,#36819,#4618,.T.);
#50269=EDGE_CURVE('',#39638,#39621,#4619,.T.);
#50270=EDGE_CURVE('',#39620,#39639,#4620,.T.);
#50271=EDGE_CURVE('',#39622,#39627,#4621,.T.);
#50272=EDGE_CURVE('',#39626,#39623,#4622,.T.);
#50273=EDGE_CURVE('',#39666,#39649,#4623,.T.);
#50274=EDGE_CURVE('',#39648,#39667,#4624,.T.);
#50275=EDGE_CURVE('',#39650,#39655,#4625,.T.);
#50276=EDGE_CURVE('',#39654,#39651,#4626,.T.);
#50277=EDGE_CURVE('',#39694,#39677,#4627,.T.);
#50278=EDGE_CURVE('',#39676,#39695,#4628,.T.);
#50279=EDGE_CURVE('',#39678,#39683,#4629,.T.);
#50280=EDGE_CURVE('',#39682,#39679,#4630,.T.);
#50281=EDGE_CURVE('',#39722,#39705,#4631,.T.);
#50282=EDGE_CURVE('',#39704,#39723,#4632,.T.);
#50283=EDGE_CURVE('',#39706,#39711,#4633,.T.);
#50284=EDGE_CURVE('',#39710,#39707,#4634,.T.);
#50285=EDGE_CURVE('',#39750,#39733,#4635,.T.);
#50286=EDGE_CURVE('',#39732,#39751,#4636,.T.);
#50287=EDGE_CURVE('',#39734,#39739,#4637,.T.);
#50288=EDGE_CURVE('',#39738,#39735,#4638,.T.);
#50289=EDGE_CURVE('',#39778,#39761,#4639,.T.);
#50290=EDGE_CURVE('',#39760,#39779,#4640,.T.);
#50291=EDGE_CURVE('',#39762,#39767,#4641,.T.);
#50292=EDGE_CURVE('',#39766,#39763,#4642,.T.);
#50293=EDGE_CURVE('',#39806,#39789,#4643,.T.);
#50294=EDGE_CURVE('',#39788,#39807,#4644,.T.);
#50295=EDGE_CURVE('',#39790,#39795,#4645,.T.);
#50296=EDGE_CURVE('',#39794,#39791,#4646,.T.);
#50297=EDGE_CURVE('',#39834,#39817,#4647,.T.);
#50298=EDGE_CURVE('',#39816,#39835,#4648,.T.);
#50299=EDGE_CURVE('',#39818,#39823,#4649,.T.);
#50300=EDGE_CURVE('',#39822,#39819,#4650,.T.);
#50301=EDGE_CURVE('',#39862,#39845,#4651,.T.);
#50302=EDGE_CURVE('',#39844,#39863,#4652,.T.);
#50303=EDGE_CURVE('',#39846,#39851,#4653,.T.);
#50304=EDGE_CURVE('',#39850,#39847,#4654,.T.);
#50305=EDGE_CURVE('',#39890,#39873,#4655,.T.);
#50306=EDGE_CURVE('',#39872,#39891,#4656,.T.);
#50307=EDGE_CURVE('',#39874,#39879,#4657,.T.);
#50308=EDGE_CURVE('',#39878,#39875,#4658,.T.);
#50309=EDGE_CURVE('',#39918,#39901,#4659,.T.);
#50310=EDGE_CURVE('',#39900,#39919,#4660,.T.);
#50311=EDGE_CURVE('',#39902,#39907,#4661,.T.);
#50312=EDGE_CURVE('',#39906,#39903,#4662,.T.);
#50313=EDGE_CURVE('',#39946,#39929,#4663,.T.);
#50314=EDGE_CURVE('',#39928,#39947,#4664,.T.);
#50315=EDGE_CURVE('',#39930,#39935,#4665,.T.);
#50316=EDGE_CURVE('',#39934,#39931,#4666,.T.);
#50317=EDGE_CURVE('',#39974,#39957,#4667,.T.);
#50318=EDGE_CURVE('',#39956,#39975,#4668,.T.);
#50319=EDGE_CURVE('',#39958,#39963,#4669,.T.);
#50320=EDGE_CURVE('',#39962,#39959,#4670,.T.);
#50321=EDGE_CURVE('',#40002,#39985,#4671,.T.);
#50322=EDGE_CURVE('',#39984,#40003,#4672,.T.);
#50323=EDGE_CURVE('',#39986,#39991,#4673,.T.);
#50324=EDGE_CURVE('',#39990,#39987,#4674,.T.);
#50325=EDGE_CURVE('',#40026,#36818,#4675,.T.);
#50326=EDGE_CURVE('',#36812,#40027,#4676,.T.);
#50327=EDGE_CURVE('',#36817,#40015,#4677,.T.);
#50328=EDGE_CURVE('',#40014,#36811,#4678,.T.);
#50329=EDGE_CURVE('',#40054,#40037,#4679,.T.);
#50330=EDGE_CURVE('',#40036,#40055,#4680,.T.);
#50331=EDGE_CURVE('',#40038,#40043,#4681,.T.);
#50332=EDGE_CURVE('',#40042,#40039,#4682,.T.);
#50333=EDGE_CURVE('',#40082,#40065,#4683,.T.);
#50334=EDGE_CURVE('',#40064,#40083,#4684,.T.);
#50335=EDGE_CURVE('',#40066,#40071,#4685,.T.);
#50336=EDGE_CURVE('',#40070,#40067,#4686,.T.);
#50337=EDGE_CURVE('',#40110,#40093,#4687,.T.);
#50338=EDGE_CURVE('',#40092,#40111,#4688,.T.);
#50339=EDGE_CURVE('',#40094,#40099,#4689,.T.);
#50340=EDGE_CURVE('',#40098,#40095,#4690,.T.);
#50341=EDGE_CURVE('',#40138,#40121,#4691,.T.);
#50342=EDGE_CURVE('',#40120,#40139,#4692,.T.);
#50343=EDGE_CURVE('',#40122,#40127,#4693,.T.);
#50344=EDGE_CURVE('',#40126,#40123,#4694,.T.);
#50345=EDGE_CURVE('',#40166,#40149,#4695,.T.);
#50346=EDGE_CURVE('',#40148,#40167,#4696,.T.);
#50347=EDGE_CURVE('',#40150,#40155,#4697,.T.);
#50348=EDGE_CURVE('',#40154,#40151,#4698,.T.);
#50349=EDGE_CURVE('',#40194,#40177,#4699,.T.);
#50350=EDGE_CURVE('',#40176,#40195,#4700,.T.);
#50351=EDGE_CURVE('',#40178,#40183,#4701,.T.);
#50352=EDGE_CURVE('',#40182,#40179,#4702,.T.);
#50353=EDGE_CURVE('',#40222,#40205,#4703,.T.);
#50354=EDGE_CURVE('',#40204,#40223,#4704,.T.);
#50355=EDGE_CURVE('',#40206,#40211,#4705,.T.);
#50356=EDGE_CURVE('',#40210,#40207,#4706,.T.);
#50357=EDGE_CURVE('',#40250,#40233,#4707,.T.);
#50358=EDGE_CURVE('',#40232,#40251,#4708,.T.);
#50359=EDGE_CURVE('',#40234,#40239,#4709,.T.);
#50360=EDGE_CURVE('',#40238,#40235,#4710,.T.);
#50361=EDGE_CURVE('',#40278,#40261,#4711,.T.);
#50362=EDGE_CURVE('',#40260,#40279,#4712,.T.);
#50363=EDGE_CURVE('',#40262,#40267,#4713,.T.);
#50364=EDGE_CURVE('',#40266,#40263,#4714,.T.);
#50365=EDGE_CURVE('',#40306,#40289,#4715,.T.);
#50366=EDGE_CURVE('',#40288,#40307,#4716,.T.);
#50367=EDGE_CURVE('',#40290,#40295,#4717,.T.);
#50368=EDGE_CURVE('',#40294,#40291,#4718,.T.);
#50369=EDGE_CURVE('',#40334,#40317,#4719,.T.);
#50370=EDGE_CURVE('',#40316,#40335,#4720,.T.);
#50371=EDGE_CURVE('',#40318,#40323,#4721,.T.);
#50372=EDGE_CURVE('',#40322,#40319,#4722,.T.);
#50373=EDGE_CURVE('',#40362,#40345,#4723,.T.);
#50374=EDGE_CURVE('',#40344,#40363,#4724,.T.);
#50375=EDGE_CURVE('',#40346,#40351,#4725,.T.);
#50376=EDGE_CURVE('',#40350,#40347,#4726,.T.);
#50377=EDGE_CURVE('',#40390,#40373,#4727,.T.);
#50378=EDGE_CURVE('',#40372,#40391,#4728,.T.);
#50379=EDGE_CURVE('',#40374,#40379,#4729,.T.);
#50380=EDGE_CURVE('',#40378,#40375,#4730,.T.);
#50381=EDGE_CURVE('',#40418,#40401,#4731,.T.);
#50382=EDGE_CURVE('',#40400,#40419,#4732,.T.);
#50383=EDGE_CURVE('',#40402,#40407,#4733,.T.);
#50384=EDGE_CURVE('',#40406,#40403,#4734,.T.);
#50385=EDGE_CURVE('',#38811,#38733,#1182,.T.);
#50386=EDGE_CURVE('',#38728,#38810,#31778,.T.);
#50387=EDGE_CURVE('',#38727,#38809,#31779,.T.);
#50388=EDGE_CURVE('',#38800,#38735,#31780,.T.);
#50389=EDGE_CURVE('',#38724,#38808,#31781,.T.);
#50390=EDGE_CURVE('',#38801,#36849,#31782,.T.);
#50391=EDGE_CURVE('',#38723,#38807,#31783,.T.);
#50392=EDGE_CURVE('',#38802,#36848,#31784,.T.);
#50393=EDGE_CURVE('',#38721,#38806,#1183,.T.);
#50394=EDGE_CURVE('',#38785,#36847,#31785,.T.);
#50395=EDGE_CURVE('',#38716,#38805,#31786,.T.);
#50396=EDGE_CURVE('',#38786,#36846,#31787,.T.);
#50397=EDGE_CURVE('',#37366,#38804,#31788,.T.);
#50398=EDGE_CURVE('',#38791,#36845,#31789,.T.);
#50399=EDGE_CURVE('',#37367,#38803,#31790,.T.);
#50400=EDGE_CURVE('',#38792,#36844,#31791,.T.);
#50401=EDGE_CURVE('',#37368,#38784,#31792,.T.);
#50402=EDGE_CURVE('',#38793,#38754,#31793,.T.);
#50403=EDGE_CURVE('',#37369,#38787,#31794,.T.);
#50404=EDGE_CURVE('',#38794,#38750,#1184,.T.);
#50405=EDGE_CURVE('',#37370,#38790,#31795,.T.);
#50406=EDGE_CURVE('',#38795,#38749,#31796,.T.);
#50407=EDGE_CURVE('',#37371,#38789,#31797,.T.);
#50408=EDGE_CURVE('',#38796,#38746,#31798,.T.);
#50409=EDGE_CURVE('',#38737,#38788,#31799,.T.);
#50410=EDGE_CURVE('',#38797,#38745,#31800,.T.);
#50411=EDGE_CURVE('',#38738,#38799,#1185,.T.);
#50412=EDGE_CURVE('',#38798,#38742,#31801,.T.);
#50413=EDGE_CURVE('',#38839,#38713,#1186,.T.);
#50414=EDGE_CURVE('',#38708,#38838,#31802,.T.);
#50415=EDGE_CURVE('',#38707,#38837,#31803,.T.);
#50416=EDGE_CURVE('',#38828,#38715,#31804,.T.);
#50417=EDGE_CURVE('',#38704,#38836,#31805,.T.);
#50418=EDGE_CURVE('',#38829,#36855,#31806,.T.);
#50419=EDGE_CURVE('',#38703,#38835,#31807,.T.);
#50420=EDGE_CURVE('',#38830,#36854,#31808,.T.);
#50421=EDGE_CURVE('',#38701,#38834,#1187,.T.);
#50422=EDGE_CURVE('',#38813,#36853,#31809,.T.);
#50423=EDGE_CURVE('',#38696,#38833,#31810,.T.);
#50424=EDGE_CURVE('',#38814,#36852,#31811,.T.);
#50425=EDGE_CURVE('',#37360,#38832,#31812,.T.);
#50426=EDGE_CURVE('',#38819,#36851,#31813,.T.);
#50427=EDGE_CURVE('',#37361,#38831,#31814,.T.);
#50428=EDGE_CURVE('',#38820,#36850,#31815,.T.);
#50429=EDGE_CURVE('',#37362,#38812,#31816,.T.);
#50430=EDGE_CURVE('',#38821,#38734,#31817,.T.);
#50431=EDGE_CURVE('',#37363,#38815,#31818,.T.);
#50432=EDGE_CURVE('',#38822,#38730,#1188,.T.);
#50433=EDGE_CURVE('',#37364,#38818,#31819,.T.);
#50434=EDGE_CURVE('',#38823,#38729,#31820,.T.);
#50435=EDGE_CURVE('',#37365,#38817,#31821,.T.);
#50436=EDGE_CURVE('',#38824,#38726,#31822,.T.);
#50437=EDGE_CURVE('',#38717,#38816,#31823,.T.);
#50438=EDGE_CURVE('',#38825,#38725,#31824,.T.);
#50439=EDGE_CURVE('',#38718,#38827,#1189,.T.);
#50440=EDGE_CURVE('',#38826,#38722,#31825,.T.);
#50441=EDGE_CURVE('',#38867,#38693,#1190,.T.);
#50442=EDGE_CURVE('',#38688,#38866,#31826,.T.);
#50443=EDGE_CURVE('',#38687,#38865,#31827,.T.);
#50444=EDGE_CURVE('',#38856,#38695,#31828,.T.);
#50445=EDGE_CURVE('',#38684,#38864,#31829,.T.);
#50446=EDGE_CURVE('',#38857,#36861,#31830,.T.);
#50447=EDGE_CURVE('',#38683,#38863,#31831,.T.);
#50448=EDGE_CURVE('',#38858,#36860,#31832,.T.);
#50449=EDGE_CURVE('',#38681,#38862,#1191,.T.);
#50450=EDGE_CURVE('',#38841,#36859,#31833,.T.);
#50451=EDGE_CURVE('',#38676,#38861,#31834,.T.);
#50452=EDGE_CURVE('',#38842,#36858,#31835,.T.);
#50453=EDGE_CURVE('',#37354,#38860,#31836,.T.);
#50454=EDGE_CURVE('',#38847,#36857,#31837,.T.);
#50455=EDGE_CURVE('',#37355,#38859,#31838,.T.);
#50456=EDGE_CURVE('',#38848,#36856,#31839,.T.);
#50457=EDGE_CURVE('',#37356,#38840,#31840,.T.);
#50458=EDGE_CURVE('',#38849,#38714,#31841,.T.);
#50459=EDGE_CURVE('',#37357,#38843,#31842,.T.);
#50460=EDGE_CURVE('',#38850,#38710,#1192,.T.);
#50461=EDGE_CURVE('',#37358,#38846,#31843,.T.);
#50462=EDGE_CURVE('',#38851,#38709,#31844,.T.);
#50463=EDGE_CURVE('',#37359,#38845,#31845,.T.);
#50464=EDGE_CURVE('',#38852,#38706,#31846,.T.);
#50465=EDGE_CURVE('',#38697,#38844,#31847,.T.);
#50466=EDGE_CURVE('',#38853,#38705,#31848,.T.);
#50467=EDGE_CURVE('',#38698,#38855,#1193,.T.);
#50468=EDGE_CURVE('',#38854,#38702,#31849,.T.);
#50469=EDGE_CURVE('',#38895,#38673,#1194,.T.);
#50470=EDGE_CURVE('',#38668,#38894,#31850,.T.);
#50471=EDGE_CURVE('',#38667,#38893,#31851,.T.);
#50472=EDGE_CURVE('',#38884,#38675,#31852,.T.);
#50473=EDGE_CURVE('',#38664,#38892,#31853,.T.);
#50474=EDGE_CURVE('',#38885,#36867,#31854,.T.);
#50475=EDGE_CURVE('',#38663,#38891,#31855,.T.);
#50476=EDGE_CURVE('',#38886,#36866,#31856,.T.);
#50477=EDGE_CURVE('',#38661,#38890,#1195,.T.);
#50478=EDGE_CURVE('',#38869,#36865,#31857,.T.);
#50479=EDGE_CURVE('',#38656,#38889,#31858,.T.);
#50480=EDGE_CURVE('',#38870,#36864,#31859,.T.);
#50481=EDGE_CURVE('',#37348,#38888,#31860,.T.);
#50482=EDGE_CURVE('',#38875,#36863,#31861,.T.);
#50483=EDGE_CURVE('',#37349,#38887,#31862,.T.);
#50484=EDGE_CURVE('',#38876,#36862,#31863,.T.);
#50485=EDGE_CURVE('',#37350,#38868,#31864,.T.);
#50486=EDGE_CURVE('',#38877,#38694,#31865,.T.);
#50487=EDGE_CURVE('',#37351,#38871,#31866,.T.);
#50488=EDGE_CURVE('',#38878,#38690,#1196,.T.);
#50489=EDGE_CURVE('',#37352,#38874,#31867,.T.);
#50490=EDGE_CURVE('',#38879,#38689,#31868,.T.);
#50491=EDGE_CURVE('',#37353,#38873,#31869,.T.);
#50492=EDGE_CURVE('',#38880,#38686,#31870,.T.);
#50493=EDGE_CURVE('',#38677,#38872,#31871,.T.);
#50494=EDGE_CURVE('',#38881,#38685,#31872,.T.);
#50495=EDGE_CURVE('',#38678,#38883,#1197,.T.);
#50496=EDGE_CURVE('',#38882,#38682,#31873,.T.);
#50497=EDGE_CURVE('',#38923,#38653,#1198,.T.);
#50498=EDGE_CURVE('',#38648,#38922,#31874,.T.);
#50499=EDGE_CURVE('',#38647,#38921,#31875,.T.);
#50500=EDGE_CURVE('',#38912,#38655,#31876,.T.);
#50501=EDGE_CURVE('',#38644,#38920,#31877,.T.);
#50502=EDGE_CURVE('',#38913,#36873,#31878,.T.);
#50503=EDGE_CURVE('',#38643,#38919,#31879,.T.);
#50504=EDGE_CURVE('',#38914,#36872,#31880,.T.);
#50505=EDGE_CURVE('',#38641,#38918,#1199,.T.);
#50506=EDGE_CURVE('',#38897,#36871,#31881,.T.);
#50507=EDGE_CURVE('',#38636,#38917,#31882,.T.);
#50508=EDGE_CURVE('',#38898,#36870,#31883,.T.);
#50509=EDGE_CURVE('',#37342,#38916,#31884,.T.);
#50510=EDGE_CURVE('',#38903,#36869,#31885,.T.);
#50511=EDGE_CURVE('',#37343,#38915,#31886,.T.);
#50512=EDGE_CURVE('',#38904,#36868,#31887,.T.);
#50513=EDGE_CURVE('',#37344,#38896,#31888,.T.);
#50514=EDGE_CURVE('',#38905,#38674,#31889,.T.);
#50515=EDGE_CURVE('',#37345,#38899,#31890,.T.);
#50516=EDGE_CURVE('',#38906,#38670,#1200,.T.);
#50517=EDGE_CURVE('',#37346,#38902,#31891,.T.);
#50518=EDGE_CURVE('',#38907,#38669,#31892,.T.);
#50519=EDGE_CURVE('',#37347,#38901,#31893,.T.);
#50520=EDGE_CURVE('',#38908,#38666,#31894,.T.);
#50521=EDGE_CURVE('',#38657,#38900,#31895,.T.);
#50522=EDGE_CURVE('',#38909,#38665,#31896,.T.);
#50523=EDGE_CURVE('',#38658,#38911,#1201,.T.);
#50524=EDGE_CURVE('',#38910,#38662,#31897,.T.);
#50525=EDGE_CURVE('',#38951,#38633,#1202,.T.);
#50526=EDGE_CURVE('',#38628,#38950,#31898,.T.);
#50527=EDGE_CURVE('',#38627,#38949,#31899,.T.);
#50528=EDGE_CURVE('',#38940,#38635,#31900,.T.);
#50529=EDGE_CURVE('',#38624,#38948,#31901,.T.);
#50530=EDGE_CURVE('',#38941,#36879,#31902,.T.);
#50531=EDGE_CURVE('',#38623,#38947,#31903,.T.);
#50532=EDGE_CURVE('',#38942,#36878,#31904,.T.);
#50533=EDGE_CURVE('',#38621,#38946,#1203,.T.);
#50534=EDGE_CURVE('',#38925,#36877,#31905,.T.);
#50535=EDGE_CURVE('',#38616,#38945,#31906,.T.);
#50536=EDGE_CURVE('',#38926,#36876,#31907,.T.);
#50537=EDGE_CURVE('',#37336,#38944,#31908,.T.);
#50538=EDGE_CURVE('',#38931,#36875,#31909,.T.);
#50539=EDGE_CURVE('',#37337,#38943,#31910,.T.);
#50540=EDGE_CURVE('',#38932,#36874,#31911,.T.);
#50541=EDGE_CURVE('',#37338,#38924,#31912,.T.);
#50542=EDGE_CURVE('',#38933,#38654,#31913,.T.);
#50543=EDGE_CURVE('',#37339,#38927,#31914,.T.);
#50544=EDGE_CURVE('',#38934,#38650,#1204,.T.);
#50545=EDGE_CURVE('',#37340,#38930,#31915,.T.);
#50546=EDGE_CURVE('',#38935,#38649,#31916,.T.);
#50547=EDGE_CURVE('',#37341,#38929,#31917,.T.);
#50548=EDGE_CURVE('',#38936,#38646,#31918,.T.);
#50549=EDGE_CURVE('',#38637,#38928,#31919,.T.);
#50550=EDGE_CURVE('',#38937,#38645,#31920,.T.);
#50551=EDGE_CURVE('',#38638,#38939,#1205,.T.);
#50552=EDGE_CURVE('',#38938,#38642,#31921,.T.);
#50553=EDGE_CURVE('',#38979,#38613,#1206,.T.);
#50554=EDGE_CURVE('',#38608,#38978,#31922,.T.);
#50555=EDGE_CURVE('',#38607,#38977,#31923,.T.);
#50556=EDGE_CURVE('',#38968,#38615,#31924,.T.);
#50557=EDGE_CURVE('',#38604,#38976,#31925,.T.);
#50558=EDGE_CURVE('',#38969,#36885,#31926,.T.);
#50559=EDGE_CURVE('',#38603,#38975,#31927,.T.);
#50560=EDGE_CURVE('',#38970,#36884,#31928,.T.);
#50561=EDGE_CURVE('',#38601,#38974,#1207,.T.);
#50562=EDGE_CURVE('',#38953,#36883,#31929,.T.);
#50563=EDGE_CURVE('',#38596,#38973,#31930,.T.);
#50564=EDGE_CURVE('',#38954,#36882,#31931,.T.);
#50565=EDGE_CURVE('',#37330,#38972,#31932,.T.);
#50566=EDGE_CURVE('',#38959,#36881,#31933,.T.);
#50567=EDGE_CURVE('',#37331,#38971,#31934,.T.);
#50568=EDGE_CURVE('',#38960,#36880,#31935,.T.);
#50569=EDGE_CURVE('',#37332,#38952,#31936,.T.);
#50570=EDGE_CURVE('',#38961,#38634,#31937,.T.);
#50571=EDGE_CURVE('',#37333,#38955,#31938,.T.);
#50572=EDGE_CURVE('',#38962,#38630,#1208,.T.);
#50573=EDGE_CURVE('',#37334,#38958,#31939,.T.);
#50574=EDGE_CURVE('',#38963,#38629,#31940,.T.);
#50575=EDGE_CURVE('',#37335,#38957,#31941,.T.);
#50576=EDGE_CURVE('',#38964,#38626,#31942,.T.);
#50577=EDGE_CURVE('',#38617,#38956,#31943,.T.);
#50578=EDGE_CURVE('',#38965,#38625,#31944,.T.);
#50579=EDGE_CURVE('',#38618,#38967,#1209,.T.);
#50580=EDGE_CURVE('',#38966,#38622,#31945,.T.);
#50581=EDGE_CURVE('',#39007,#38593,#1210,.T.);
#50582=EDGE_CURVE('',#38588,#39006,#31946,.T.);
#50583=EDGE_CURVE('',#38587,#39005,#31947,.T.);
#50584=EDGE_CURVE('',#38996,#38595,#31948,.T.);
#50585=EDGE_CURVE('',#38584,#39004,#31949,.T.);
#50586=EDGE_CURVE('',#38997,#36891,#31950,.T.);
#50587=EDGE_CURVE('',#38583,#39003,#31951,.T.);
#50588=EDGE_CURVE('',#38998,#36890,#31952,.T.);
#50589=EDGE_CURVE('',#38581,#39002,#1211,.T.);
#50590=EDGE_CURVE('',#38981,#36889,#31953,.T.);
#50591=EDGE_CURVE('',#38576,#39001,#31954,.T.);
#50592=EDGE_CURVE('',#38982,#36888,#31955,.T.);
#50593=EDGE_CURVE('',#37324,#39000,#31956,.T.);
#50594=EDGE_CURVE('',#38987,#36887,#31957,.T.);
#50595=EDGE_CURVE('',#37325,#38999,#31958,.T.);
#50596=EDGE_CURVE('',#38988,#36886,#31959,.T.);
#50597=EDGE_CURVE('',#37326,#38980,#31960,.T.);
#50598=EDGE_CURVE('',#38989,#38614,#31961,.T.);
#50599=EDGE_CURVE('',#37327,#38983,#31962,.T.);
#50600=EDGE_CURVE('',#38990,#38610,#1212,.T.);
#50601=EDGE_CURVE('',#37328,#38986,#31963,.T.);
#50602=EDGE_CURVE('',#38991,#38609,#31964,.T.);
#50603=EDGE_CURVE('',#37329,#38985,#31965,.T.);
#50604=EDGE_CURVE('',#38992,#38606,#31966,.T.);
#50605=EDGE_CURVE('',#38597,#38984,#31967,.T.);
#50606=EDGE_CURVE('',#38993,#38605,#31968,.T.);
#50607=EDGE_CURVE('',#38598,#38995,#1213,.T.);
#50608=EDGE_CURVE('',#38994,#38602,#31969,.T.);
#50609=EDGE_CURVE('',#39035,#38573,#1214,.T.);
#50610=EDGE_CURVE('',#38568,#39034,#31970,.T.);
#50611=EDGE_CURVE('',#38567,#39033,#31971,.T.);
#50612=EDGE_CURVE('',#39024,#38575,#31972,.T.);
#50613=EDGE_CURVE('',#38564,#39032,#31973,.T.);
#50614=EDGE_CURVE('',#39025,#36897,#31974,.T.);
#50615=EDGE_CURVE('',#38563,#39031,#31975,.T.);
#50616=EDGE_CURVE('',#39026,#36896,#31976,.T.);
#50617=EDGE_CURVE('',#38561,#39030,#1215,.T.);
#50618=EDGE_CURVE('',#39009,#36895,#31977,.T.);
#50619=EDGE_CURVE('',#38556,#39029,#31978,.T.);
#50620=EDGE_CURVE('',#39010,#36894,#31979,.T.);
#50621=EDGE_CURVE('',#37318,#39028,#31980,.T.);
#50622=EDGE_CURVE('',#39015,#36893,#31981,.T.);
#50623=EDGE_CURVE('',#37319,#39027,#31982,.T.);
#50624=EDGE_CURVE('',#39016,#36892,#31983,.T.);
#50625=EDGE_CURVE('',#37320,#39008,#31984,.T.);
#50626=EDGE_CURVE('',#39017,#38594,#31985,.T.);
#50627=EDGE_CURVE('',#37321,#39011,#31986,.T.);
#50628=EDGE_CURVE('',#39018,#38590,#1216,.T.);
#50629=EDGE_CURVE('',#37322,#39014,#31987,.T.);
#50630=EDGE_CURVE('',#39019,#38589,#31988,.T.);
#50631=EDGE_CURVE('',#37323,#39013,#31989,.T.);
#50632=EDGE_CURVE('',#39020,#38586,#31990,.T.);
#50633=EDGE_CURVE('',#38577,#39012,#31991,.T.);
#50634=EDGE_CURVE('',#39021,#38585,#31992,.T.);
#50635=EDGE_CURVE('',#38578,#39023,#1217,.T.);
#50636=EDGE_CURVE('',#39022,#38582,#31993,.T.);
#50637=EDGE_CURVE('',#39063,#38553,#1218,.T.);
#50638=EDGE_CURVE('',#38548,#39062,#31994,.T.);
#50639=EDGE_CURVE('',#38547,#39061,#31995,.T.);
#50640=EDGE_CURVE('',#39052,#38555,#31996,.T.);
#50641=EDGE_CURVE('',#38544,#39060,#31997,.T.);
#50642=EDGE_CURVE('',#39053,#36903,#31998,.T.);
#50643=EDGE_CURVE('',#38543,#39059,#31999,.T.);
#50644=EDGE_CURVE('',#39054,#36902,#32000,.T.);
#50645=EDGE_CURVE('',#38541,#39058,#1219,.T.);
#50646=EDGE_CURVE('',#39037,#36901,#32001,.T.);
#50647=EDGE_CURVE('',#38536,#39057,#32002,.T.);
#50648=EDGE_CURVE('',#39038,#36900,#32003,.T.);
#50649=EDGE_CURVE('',#37312,#39056,#32004,.T.);
#50650=EDGE_CURVE('',#39043,#36899,#32005,.T.);
#50651=EDGE_CURVE('',#37313,#39055,#32006,.T.);
#50652=EDGE_CURVE('',#39044,#36898,#32007,.T.);
#50653=EDGE_CURVE('',#37314,#39036,#32008,.T.);
#50654=EDGE_CURVE('',#39045,#38574,#32009,.T.);
#50655=EDGE_CURVE('',#37315,#39039,#32010,.T.);
#50656=EDGE_CURVE('',#39046,#38570,#1220,.T.);
#50657=EDGE_CURVE('',#37316,#39042,#32011,.T.);
#50658=EDGE_CURVE('',#39047,#38569,#32012,.T.);
#50659=EDGE_CURVE('',#37317,#39041,#32013,.T.);
#50660=EDGE_CURVE('',#39048,#38566,#32014,.T.);
#50661=EDGE_CURVE('',#38557,#39040,#32015,.T.);
#50662=EDGE_CURVE('',#39049,#38565,#32016,.T.);
#50663=EDGE_CURVE('',#38558,#39051,#1221,.T.);
#50664=EDGE_CURVE('',#39050,#38562,#32017,.T.);
#50665=EDGE_CURVE('',#39091,#38533,#1222,.T.);
#50666=EDGE_CURVE('',#38528,#39090,#32018,.T.);
#50667=EDGE_CURVE('',#38527,#39089,#32019,.T.);
#50668=EDGE_CURVE('',#39080,#38535,#32020,.T.);
#50669=EDGE_CURVE('',#38524,#39088,#32021,.T.);
#50670=EDGE_CURVE('',#39081,#36909,#32022,.T.);
#50671=EDGE_CURVE('',#38523,#39087,#32023,.T.);
#50672=EDGE_CURVE('',#39082,#36908,#32024,.T.);
#50673=EDGE_CURVE('',#38521,#39086,#1223,.T.);
#50674=EDGE_CURVE('',#39065,#36907,#32025,.T.);
#50675=EDGE_CURVE('',#38516,#39085,#32026,.T.);
#50676=EDGE_CURVE('',#39066,#36906,#32027,.T.);
#50677=EDGE_CURVE('',#37306,#39084,#32028,.T.);
#50678=EDGE_CURVE('',#39071,#36905,#32029,.T.);
#50679=EDGE_CURVE('',#37307,#39083,#32030,.T.);
#50680=EDGE_CURVE('',#39072,#36904,#32031,.T.);
#50681=EDGE_CURVE('',#37308,#39064,#32032,.T.);
#50682=EDGE_CURVE('',#39073,#38554,#32033,.T.);
#50683=EDGE_CURVE('',#37309,#39067,#32034,.T.);
#50684=EDGE_CURVE('',#39074,#38550,#1224,.T.);
#50685=EDGE_CURVE('',#37310,#39070,#32035,.T.);
#50686=EDGE_CURVE('',#39075,#38549,#32036,.T.);
#50687=EDGE_CURVE('',#37311,#39069,#32037,.T.);
#50688=EDGE_CURVE('',#39076,#38546,#32038,.T.);
#50689=EDGE_CURVE('',#38537,#39068,#32039,.T.);
#50690=EDGE_CURVE('',#39077,#38545,#32040,.T.);
#50691=EDGE_CURVE('',#38538,#39079,#1225,.T.);
#50692=EDGE_CURVE('',#39078,#38542,#32041,.T.);
#50693=EDGE_CURVE('',#39119,#38513,#1226,.T.);
#50694=EDGE_CURVE('',#38508,#39118,#32042,.T.);
#50695=EDGE_CURVE('',#38507,#39117,#32043,.T.);
#50696=EDGE_CURVE('',#39108,#38515,#32044,.T.);
#50697=EDGE_CURVE('',#38504,#39116,#32045,.T.);
#50698=EDGE_CURVE('',#39109,#36915,#32046,.T.);
#50699=EDGE_CURVE('',#38503,#39115,#32047,.T.);
#50700=EDGE_CURVE('',#39110,#36914,#32048,.T.);
#50701=EDGE_CURVE('',#38501,#39114,#1227,.T.);
#50702=EDGE_CURVE('',#39093,#36913,#32049,.T.);
#50703=EDGE_CURVE('',#38496,#39113,#32050,.T.);
#50704=EDGE_CURVE('',#39094,#36912,#32051,.T.);
#50705=EDGE_CURVE('',#37300,#39112,#32052,.T.);
#50706=EDGE_CURVE('',#39099,#36911,#32053,.T.);
#50707=EDGE_CURVE('',#37301,#39111,#32054,.T.);
#50708=EDGE_CURVE('',#39100,#36910,#32055,.T.);
#50709=EDGE_CURVE('',#37302,#39092,#32056,.T.);
#50710=EDGE_CURVE('',#39101,#38534,#32057,.T.);
#50711=EDGE_CURVE('',#37303,#39095,#32058,.T.);
#50712=EDGE_CURVE('',#39102,#38530,#1228,.T.);
#50713=EDGE_CURVE('',#37304,#39098,#32059,.T.);
#50714=EDGE_CURVE('',#39103,#38529,#32060,.T.);
#50715=EDGE_CURVE('',#37305,#39097,#32061,.T.);
#50716=EDGE_CURVE('',#39104,#38526,#32062,.T.);
#50717=EDGE_CURVE('',#38517,#39096,#32063,.T.);
#50718=EDGE_CURVE('',#39105,#38525,#32064,.T.);
#50719=EDGE_CURVE('',#38518,#39107,#1229,.T.);
#50720=EDGE_CURVE('',#39106,#38522,#32065,.T.);
#50721=EDGE_CURVE('',#39147,#38493,#1230,.T.);
#50722=EDGE_CURVE('',#38488,#39146,#32066,.T.);
#50723=EDGE_CURVE('',#38487,#39145,#32067,.T.);
#50724=EDGE_CURVE('',#39136,#38495,#32068,.T.);
#50725=EDGE_CURVE('',#38484,#39144,#32069,.T.);
#50726=EDGE_CURVE('',#39137,#36921,#32070,.T.);
#50727=EDGE_CURVE('',#38483,#39143,#32071,.T.);
#50728=EDGE_CURVE('',#39138,#36920,#32072,.T.);
#50729=EDGE_CURVE('',#38481,#39142,#1231,.T.);
#50730=EDGE_CURVE('',#39121,#36919,#32073,.T.);
#50731=EDGE_CURVE('',#38476,#39141,#32074,.T.);
#50732=EDGE_CURVE('',#39122,#36918,#32075,.T.);
#50733=EDGE_CURVE('',#37294,#39140,#32076,.T.);
#50734=EDGE_CURVE('',#39127,#36917,#32077,.T.);
#50735=EDGE_CURVE('',#37295,#39139,#32078,.T.);
#50736=EDGE_CURVE('',#39128,#36916,#32079,.T.);
#50737=EDGE_CURVE('',#37296,#39120,#32080,.T.);
#50738=EDGE_CURVE('',#39129,#38514,#32081,.T.);
#50739=EDGE_CURVE('',#37297,#39123,#32082,.T.);
#50740=EDGE_CURVE('',#39130,#38510,#1232,.T.);
#50741=EDGE_CURVE('',#37298,#39126,#32083,.T.);
#50742=EDGE_CURVE('',#39131,#38509,#32084,.T.);
#50743=EDGE_CURVE('',#37299,#39125,#32085,.T.);
#50744=EDGE_CURVE('',#39132,#38506,#32086,.T.);
#50745=EDGE_CURVE('',#38497,#39124,#32087,.T.);
#50746=EDGE_CURVE('',#39133,#38505,#32088,.T.);
#50747=EDGE_CURVE('',#38498,#39135,#1233,.T.);
#50748=EDGE_CURVE('',#39134,#38502,#32089,.T.);
#50749=EDGE_CURVE('',#39175,#38473,#1234,.T.);
#50750=EDGE_CURVE('',#38468,#39174,#32090,.T.);
#50751=EDGE_CURVE('',#38467,#39173,#32091,.T.);
#50752=EDGE_CURVE('',#39164,#38475,#32092,.T.);
#50753=EDGE_CURVE('',#38464,#39172,#32093,.T.);
#50754=EDGE_CURVE('',#39165,#36927,#32094,.T.);
#50755=EDGE_CURVE('',#38463,#39171,#32095,.T.);
#50756=EDGE_CURVE('',#39166,#36926,#32096,.T.);
#50757=EDGE_CURVE('',#38461,#39170,#1235,.T.);
#50758=EDGE_CURVE('',#39149,#36925,#32097,.T.);
#50759=EDGE_CURVE('',#38456,#39169,#32098,.T.);
#50760=EDGE_CURVE('',#39150,#36924,#32099,.T.);
#50761=EDGE_CURVE('',#37288,#39168,#32100,.T.);
#50762=EDGE_CURVE('',#39155,#36923,#32101,.T.);
#50763=EDGE_CURVE('',#37289,#39167,#32102,.T.);
#50764=EDGE_CURVE('',#39156,#36922,#32103,.T.);
#50765=EDGE_CURVE('',#37290,#39148,#32104,.T.);
#50766=EDGE_CURVE('',#39157,#38494,#32105,.T.);
#50767=EDGE_CURVE('',#37291,#39151,#32106,.T.);
#50768=EDGE_CURVE('',#39158,#38490,#1236,.T.);
#50769=EDGE_CURVE('',#37292,#39154,#32107,.T.);
#50770=EDGE_CURVE('',#39159,#38489,#32108,.T.);
#50771=EDGE_CURVE('',#37293,#39153,#32109,.T.);
#50772=EDGE_CURVE('',#39160,#38486,#32110,.T.);
#50773=EDGE_CURVE('',#38477,#39152,#32111,.T.);
#50774=EDGE_CURVE('',#39161,#38485,#32112,.T.);
#50775=EDGE_CURVE('',#38478,#39163,#1237,.T.);
#50776=EDGE_CURVE('',#39162,#38482,#32113,.T.);
#50777=EDGE_CURVE('',#39203,#38453,#1238,.T.);
#50778=EDGE_CURVE('',#38448,#39202,#32114,.T.);
#50779=EDGE_CURVE('',#38447,#39201,#32115,.T.);
#50780=EDGE_CURVE('',#39192,#38455,#32116,.T.);
#50781=EDGE_CURVE('',#38444,#39200,#32117,.T.);
#50782=EDGE_CURVE('',#39193,#36933,#32118,.T.);
#50783=EDGE_CURVE('',#38443,#39199,#32119,.T.);
#50784=EDGE_CURVE('',#39194,#36932,#32120,.T.);
#50785=EDGE_CURVE('',#38441,#39198,#1239,.T.);
#50786=EDGE_CURVE('',#39177,#36931,#32121,.T.);
#50787=EDGE_CURVE('',#38436,#39197,#32122,.T.);
#50788=EDGE_CURVE('',#39178,#36930,#32123,.T.);
#50789=EDGE_CURVE('',#37282,#39196,#32124,.T.);
#50790=EDGE_CURVE('',#39183,#36929,#32125,.T.);
#50791=EDGE_CURVE('',#37283,#39195,#32126,.T.);
#50792=EDGE_CURVE('',#39184,#36928,#32127,.T.);
#50793=EDGE_CURVE('',#37284,#39176,#32128,.T.);
#50794=EDGE_CURVE('',#39185,#38474,#32129,.T.);
#50795=EDGE_CURVE('',#37285,#39179,#32130,.T.);
#50796=EDGE_CURVE('',#39186,#38470,#1240,.T.);
#50797=EDGE_CURVE('',#37286,#39182,#32131,.T.);
#50798=EDGE_CURVE('',#39187,#38469,#32132,.T.);
#50799=EDGE_CURVE('',#37287,#39181,#32133,.T.);
#50800=EDGE_CURVE('',#39188,#38466,#32134,.T.);
#50801=EDGE_CURVE('',#38457,#39180,#32135,.T.);
#50802=EDGE_CURVE('',#39189,#38465,#32136,.T.);
#50803=EDGE_CURVE('',#38458,#39191,#1241,.T.);
#50804=EDGE_CURVE('',#39190,#38462,#32137,.T.);
#50805=EDGE_CURVE('',#39231,#38433,#1242,.T.);
#50806=EDGE_CURVE('',#38428,#39230,#32138,.T.);
#50807=EDGE_CURVE('',#38427,#39229,#32139,.T.);
#50808=EDGE_CURVE('',#39220,#38435,#32140,.T.);
#50809=EDGE_CURVE('',#38424,#39228,#32141,.T.);
#50810=EDGE_CURVE('',#39221,#36939,#32142,.T.);
#50811=EDGE_CURVE('',#38423,#39227,#32143,.T.);
#50812=EDGE_CURVE('',#39222,#36938,#32144,.T.);
#50813=EDGE_CURVE('',#38421,#39226,#1243,.T.);
#50814=EDGE_CURVE('',#39205,#36937,#32145,.T.);
#50815=EDGE_CURVE('',#38416,#39225,#32146,.T.);
#50816=EDGE_CURVE('',#39206,#36936,#32147,.T.);
#50817=EDGE_CURVE('',#37276,#39224,#32148,.T.);
#50818=EDGE_CURVE('',#39211,#36935,#32149,.T.);
#50819=EDGE_CURVE('',#37277,#39223,#32150,.T.);
#50820=EDGE_CURVE('',#39212,#36934,#32151,.T.);
#50821=EDGE_CURVE('',#37278,#39204,#32152,.T.);
#50822=EDGE_CURVE('',#39213,#38454,#32153,.T.);
#50823=EDGE_CURVE('',#37279,#39207,#32154,.T.);
#50824=EDGE_CURVE('',#39214,#38450,#1244,.T.);
#50825=EDGE_CURVE('',#37280,#39210,#32155,.T.);
#50826=EDGE_CURVE('',#39215,#38449,#32156,.T.);
#50827=EDGE_CURVE('',#37281,#39209,#32157,.T.);
#50828=EDGE_CURVE('',#39216,#38446,#32158,.T.);
#50829=EDGE_CURVE('',#38437,#39208,#32159,.T.);
#50830=EDGE_CURVE('',#39217,#38445,#32160,.T.);
#50831=EDGE_CURVE('',#38438,#39219,#1245,.T.);
#50832=EDGE_CURVE('',#39218,#38442,#32161,.T.);
#50833=EDGE_CURVE('',#39259,#38413,#1246,.T.);
#50834=EDGE_CURVE('',#38408,#39258,#32162,.T.);
#50835=EDGE_CURVE('',#38407,#39257,#32163,.T.);
#50836=EDGE_CURVE('',#39248,#38415,#32164,.T.);
#50837=EDGE_CURVE('',#38404,#39256,#32165,.T.);
#50838=EDGE_CURVE('',#39249,#36945,#32166,.T.);
#50839=EDGE_CURVE('',#38403,#39255,#32167,.T.);
#50840=EDGE_CURVE('',#39250,#36944,#32168,.T.);
#50841=EDGE_CURVE('',#38401,#39254,#1247,.T.);
#50842=EDGE_CURVE('',#39233,#36943,#32169,.T.);
#50843=EDGE_CURVE('',#38396,#39253,#32170,.T.);
#50844=EDGE_CURVE('',#39234,#36942,#32171,.T.);
#50845=EDGE_CURVE('',#37270,#39252,#32172,.T.);
#50846=EDGE_CURVE('',#39239,#36941,#32173,.T.);
#50847=EDGE_CURVE('',#37271,#39251,#32174,.T.);
#50848=EDGE_CURVE('',#39240,#36940,#32175,.T.);
#50849=EDGE_CURVE('',#37272,#39232,#32176,.T.);
#50850=EDGE_CURVE('',#39241,#38434,#32177,.T.);
#50851=EDGE_CURVE('',#37273,#39235,#32178,.T.);
#50852=EDGE_CURVE('',#39242,#38430,#1248,.T.);
#50853=EDGE_CURVE('',#37274,#39238,#32179,.T.);
#50854=EDGE_CURVE('',#39243,#38429,#32180,.T.);
#50855=EDGE_CURVE('',#37275,#39237,#32181,.T.);
#50856=EDGE_CURVE('',#39244,#38426,#32182,.T.);
#50857=EDGE_CURVE('',#38417,#39236,#32183,.T.);
#50858=EDGE_CURVE('',#39245,#38425,#32184,.T.);
#50859=EDGE_CURVE('',#38418,#39247,#1249,.T.);
#50860=EDGE_CURVE('',#39246,#38422,#32185,.T.);
#50861=EDGE_CURVE('',#39287,#38393,#1250,.T.);
#50862=EDGE_CURVE('',#38388,#39286,#32186,.T.);
#50863=EDGE_CURVE('',#38387,#39285,#32187,.T.);
#50864=EDGE_CURVE('',#39276,#38395,#32188,.T.);
#50865=EDGE_CURVE('',#38384,#39284,#32189,.T.);
#50866=EDGE_CURVE('',#39277,#36951,#32190,.T.);
#50867=EDGE_CURVE('',#38383,#39283,#32191,.T.);
#50868=EDGE_CURVE('',#39278,#36950,#32192,.T.);
#50869=EDGE_CURVE('',#38381,#39282,#1251,.T.);
#50870=EDGE_CURVE('',#39261,#36949,#32193,.T.);
#50871=EDGE_CURVE('',#38376,#39281,#32194,.T.);
#50872=EDGE_CURVE('',#39262,#36948,#32195,.T.);
#50873=EDGE_CURVE('',#37264,#39280,#32196,.T.);
#50874=EDGE_CURVE('',#39267,#36947,#32197,.T.);
#50875=EDGE_CURVE('',#37265,#39279,#32198,.T.);
#50876=EDGE_CURVE('',#39268,#36946,#32199,.T.);
#50877=EDGE_CURVE('',#37266,#39260,#32200,.T.);
#50878=EDGE_CURVE('',#39269,#38414,#32201,.T.);
#50879=EDGE_CURVE('',#37267,#39263,#32202,.T.);
#50880=EDGE_CURVE('',#39270,#38410,#1252,.T.);
#50881=EDGE_CURVE('',#37268,#39266,#32203,.T.);
#50882=EDGE_CURVE('',#39271,#38409,#32204,.T.);
#50883=EDGE_CURVE('',#37269,#39265,#32205,.T.);
#50884=EDGE_CURVE('',#39272,#38406,#32206,.T.);
#50885=EDGE_CURVE('',#38397,#39264,#32207,.T.);
#50886=EDGE_CURVE('',#39273,#38405,#32208,.T.);
#50887=EDGE_CURVE('',#38398,#39275,#1253,.T.);
#50888=EDGE_CURVE('',#39274,#38402,#32209,.T.);
#50889=EDGE_CURVE('',#39315,#38373,#1254,.T.);
#50890=EDGE_CURVE('',#38368,#39314,#32210,.T.);
#50891=EDGE_CURVE('',#38367,#39313,#32211,.T.);
#50892=EDGE_CURVE('',#39304,#38375,#32212,.T.);
#50893=EDGE_CURVE('',#38364,#39312,#32213,.T.);
#50894=EDGE_CURVE('',#39305,#36957,#32214,.T.);
#50895=EDGE_CURVE('',#38363,#39311,#32215,.T.);
#50896=EDGE_CURVE('',#39306,#36956,#32216,.T.);
#50897=EDGE_CURVE('',#38361,#39310,#1255,.T.);
#50898=EDGE_CURVE('',#39289,#36955,#32217,.T.);
#50899=EDGE_CURVE('',#38356,#39309,#32218,.T.);
#50900=EDGE_CURVE('',#39290,#36954,#32219,.T.);
#50901=EDGE_CURVE('',#37258,#39308,#32220,.T.);
#50902=EDGE_CURVE('',#39295,#36953,#32221,.T.);
#50903=EDGE_CURVE('',#37259,#39307,#32222,.T.);
#50904=EDGE_CURVE('',#39296,#36952,#32223,.T.);
#50905=EDGE_CURVE('',#37260,#39288,#32224,.T.);
#50906=EDGE_CURVE('',#39297,#38394,#32225,.T.);
#50907=EDGE_CURVE('',#37261,#39291,#32226,.T.);
#50908=EDGE_CURVE('',#39298,#38390,#1256,.T.);
#50909=EDGE_CURVE('',#37262,#39294,#32227,.T.);
#50910=EDGE_CURVE('',#39299,#38389,#32228,.T.);
#50911=EDGE_CURVE('',#37263,#39293,#32229,.T.);
#50912=EDGE_CURVE('',#39300,#38386,#32230,.T.);
#50913=EDGE_CURVE('',#38377,#39292,#32231,.T.);
#50914=EDGE_CURVE('',#39301,#38385,#32232,.T.);
#50915=EDGE_CURVE('',#38378,#39303,#1257,.T.);
#50916=EDGE_CURVE('',#39302,#38382,#32233,.T.);
#50917=EDGE_CURVE('',#39343,#38353,#1258,.T.);
#50918=EDGE_CURVE('',#38348,#39342,#32234,.T.);
#50919=EDGE_CURVE('',#38347,#39341,#32235,.T.);
#50920=EDGE_CURVE('',#39332,#38355,#32236,.T.);
#50921=EDGE_CURVE('',#38344,#39340,#32237,.T.);
#50922=EDGE_CURVE('',#39333,#36963,#32238,.T.);
#50923=EDGE_CURVE('',#38343,#39339,#32239,.T.);
#50924=EDGE_CURVE('',#39334,#36962,#32240,.T.);
#50925=EDGE_CURVE('',#38341,#39338,#1259,.T.);
#50926=EDGE_CURVE('',#39317,#36961,#32241,.T.);
#50927=EDGE_CURVE('',#38336,#39337,#32242,.T.);
#50928=EDGE_CURVE('',#39318,#36960,#32243,.T.);
#50929=EDGE_CURVE('',#37252,#39336,#32244,.T.);
#50930=EDGE_CURVE('',#39323,#36959,#32245,.T.);
#50931=EDGE_CURVE('',#37253,#39335,#32246,.T.);
#50932=EDGE_CURVE('',#39324,#36958,#32247,.T.);
#50933=EDGE_CURVE('',#37254,#39316,#32248,.T.);
#50934=EDGE_CURVE('',#39325,#38374,#32249,.T.);
#50935=EDGE_CURVE('',#37255,#39319,#32250,.T.);
#50936=EDGE_CURVE('',#39326,#38370,#1260,.T.);
#50937=EDGE_CURVE('',#37256,#39322,#32251,.T.);
#50938=EDGE_CURVE('',#39327,#38369,#32252,.T.);
#50939=EDGE_CURVE('',#37257,#39321,#32253,.T.);
#50940=EDGE_CURVE('',#39328,#38366,#32254,.T.);
#50941=EDGE_CURVE('',#38357,#39320,#32255,.T.);
#50942=EDGE_CURVE('',#39329,#38365,#32256,.T.);
#50943=EDGE_CURVE('',#38358,#39331,#1261,.T.);
#50944=EDGE_CURVE('',#39330,#38362,#32257,.T.);
#50945=EDGE_CURVE('',#39371,#38333,#1262,.T.);
#50946=EDGE_CURVE('',#38328,#39370,#32258,.T.);
#50947=EDGE_CURVE('',#38327,#39369,#32259,.T.);
#50948=EDGE_CURVE('',#39360,#38335,#32260,.T.);
#50949=EDGE_CURVE('',#38324,#39368,#32261,.T.);
#50950=EDGE_CURVE('',#39361,#36969,#32262,.T.);
#50951=EDGE_CURVE('',#38323,#39367,#32263,.T.);
#50952=EDGE_CURVE('',#39362,#36968,#32264,.T.);
#50953=EDGE_CURVE('',#38321,#39366,#1263,.T.);
#50954=EDGE_CURVE('',#39345,#36967,#32265,.T.);
#50955=EDGE_CURVE('',#38316,#39365,#32266,.T.);
#50956=EDGE_CURVE('',#39346,#36966,#32267,.T.);
#50957=EDGE_CURVE('',#37246,#39364,#32268,.T.);
#50958=EDGE_CURVE('',#39351,#36965,#32269,.T.);
#50959=EDGE_CURVE('',#37247,#39363,#32270,.T.);
#50960=EDGE_CURVE('',#39352,#36964,#32271,.T.);
#50961=EDGE_CURVE('',#37248,#39344,#32272,.T.);
#50962=EDGE_CURVE('',#39353,#38354,#32273,.T.);
#50963=EDGE_CURVE('',#37249,#39347,#32274,.T.);
#50964=EDGE_CURVE('',#39354,#38350,#1264,.T.);
#50965=EDGE_CURVE('',#37250,#39350,#32275,.T.);
#50966=EDGE_CURVE('',#39355,#38349,#32276,.T.);
#50967=EDGE_CURVE('',#37251,#39349,#32277,.T.);
#50968=EDGE_CURVE('',#39356,#38346,#32278,.T.);
#50969=EDGE_CURVE('',#38337,#39348,#32279,.T.);
#50970=EDGE_CURVE('',#39357,#38345,#32280,.T.);
#50971=EDGE_CURVE('',#38338,#39359,#1265,.T.);
#50972=EDGE_CURVE('',#39358,#38342,#32281,.T.);
#50973=EDGE_CURVE('',#39399,#38313,#1266,.T.);
#50974=EDGE_CURVE('',#38308,#39398,#32282,.T.);
#50975=EDGE_CURVE('',#38307,#39397,#32283,.T.);
#50976=EDGE_CURVE('',#39388,#38315,#32284,.T.);
#50977=EDGE_CURVE('',#38304,#39396,#32285,.T.);
#50978=EDGE_CURVE('',#39389,#36975,#32286,.T.);
#50979=EDGE_CURVE('',#38303,#39395,#32287,.T.);
#50980=EDGE_CURVE('',#39390,#36974,#32288,.T.);
#50981=EDGE_CURVE('',#38301,#39394,#1267,.T.);
#50982=EDGE_CURVE('',#39373,#36973,#32289,.T.);
#50983=EDGE_CURVE('',#38296,#39393,#32290,.T.);
#50984=EDGE_CURVE('',#39374,#36972,#32291,.T.);
#50985=EDGE_CURVE('',#37240,#39392,#32292,.T.);
#50986=EDGE_CURVE('',#39379,#36971,#32293,.T.);
#50987=EDGE_CURVE('',#37241,#39391,#32294,.T.);
#50988=EDGE_CURVE('',#39380,#36970,#32295,.T.);
#50989=EDGE_CURVE('',#37242,#39372,#32296,.T.);
#50990=EDGE_CURVE('',#39381,#38334,#32297,.T.);
#50991=EDGE_CURVE('',#37243,#39375,#32298,.T.);
#50992=EDGE_CURVE('',#39382,#38330,#1268,.T.);
#50993=EDGE_CURVE('',#37244,#39378,#32299,.T.);
#50994=EDGE_CURVE('',#39383,#38329,#32300,.T.);
#50995=EDGE_CURVE('',#37245,#39377,#32301,.T.);
#50996=EDGE_CURVE('',#39384,#38326,#32302,.T.);
#50997=EDGE_CURVE('',#38317,#39376,#32303,.T.);
#50998=EDGE_CURVE('',#39385,#38325,#32304,.T.);
#50999=EDGE_CURVE('',#38318,#39387,#1269,.T.);
#51000=EDGE_CURVE('',#39386,#38322,#32305,.T.);
#51001=EDGE_CURVE('',#39427,#38293,#1270,.T.);
#51002=EDGE_CURVE('',#38288,#39426,#32306,.T.);
#51003=EDGE_CURVE('',#38287,#39425,#32307,.T.);
#51004=EDGE_CURVE('',#39416,#38295,#32308,.T.);
#51005=EDGE_CURVE('',#38284,#39424,#32309,.T.);
#51006=EDGE_CURVE('',#39417,#36981,#32310,.T.);
#51007=EDGE_CURVE('',#38283,#39423,#32311,.T.);
#51008=EDGE_CURVE('',#39418,#36980,#32312,.T.);
#51009=EDGE_CURVE('',#38281,#39422,#1271,.T.);
#51010=EDGE_CURVE('',#39401,#36979,#32313,.T.);
#51011=EDGE_CURVE('',#38276,#39421,#32314,.T.);
#51012=EDGE_CURVE('',#39402,#36978,#32315,.T.);
#51013=EDGE_CURVE('',#37234,#39420,#32316,.T.);
#51014=EDGE_CURVE('',#39407,#36977,#32317,.T.);
#51015=EDGE_CURVE('',#37235,#39419,#32318,.T.);
#51016=EDGE_CURVE('',#39408,#36976,#32319,.T.);
#51017=EDGE_CURVE('',#37236,#39400,#32320,.T.);
#51018=EDGE_CURVE('',#39409,#38314,#32321,.T.);
#51019=EDGE_CURVE('',#37237,#39403,#32322,.T.);
#51020=EDGE_CURVE('',#39410,#38310,#1272,.T.);
#51021=EDGE_CURVE('',#37238,#39406,#32323,.T.);
#51022=EDGE_CURVE('',#39411,#38309,#32324,.T.);
#51023=EDGE_CURVE('',#37239,#39405,#32325,.T.);
#51024=EDGE_CURVE('',#39412,#38306,#32326,.T.);
#51025=EDGE_CURVE('',#38297,#39404,#32327,.T.);
#51026=EDGE_CURVE('',#39413,#38305,#32328,.T.);
#51027=EDGE_CURVE('',#38298,#39415,#1273,.T.);
#51028=EDGE_CURVE('',#39414,#38302,#32329,.T.);
#51029=EDGE_CURVE('',#39455,#38273,#1274,.T.);
#51030=EDGE_CURVE('',#38268,#39454,#32330,.T.);
#51031=EDGE_CURVE('',#38267,#39453,#32331,.T.);
#51032=EDGE_CURVE('',#39444,#38275,#32332,.T.);
#51033=EDGE_CURVE('',#38264,#39452,#32333,.T.);
#51034=EDGE_CURVE('',#39445,#36987,#32334,.T.);
#51035=EDGE_CURVE('',#38263,#39451,#32335,.T.);
#51036=EDGE_CURVE('',#39446,#36986,#32336,.T.);
#51037=EDGE_CURVE('',#38261,#39450,#1275,.T.);
#51038=EDGE_CURVE('',#39429,#36985,#32337,.T.);
#51039=EDGE_CURVE('',#38256,#39449,#32338,.T.);
#51040=EDGE_CURVE('',#39430,#36984,#32339,.T.);
#51041=EDGE_CURVE('',#37228,#39448,#32340,.T.);
#51042=EDGE_CURVE('',#39435,#36983,#32341,.T.);
#51043=EDGE_CURVE('',#37229,#39447,#32342,.T.);
#51044=EDGE_CURVE('',#39436,#36982,#32343,.T.);
#51045=EDGE_CURVE('',#37230,#39428,#32344,.T.);
#51046=EDGE_CURVE('',#39437,#38294,#32345,.T.);
#51047=EDGE_CURVE('',#37231,#39431,#32346,.T.);
#51048=EDGE_CURVE('',#39438,#38290,#1276,.T.);
#51049=EDGE_CURVE('',#37232,#39434,#32347,.T.);
#51050=EDGE_CURVE('',#39439,#38289,#32348,.T.);
#51051=EDGE_CURVE('',#37233,#39433,#32349,.T.);
#51052=EDGE_CURVE('',#39440,#38286,#32350,.T.);
#51053=EDGE_CURVE('',#38277,#39432,#32351,.T.);
#51054=EDGE_CURVE('',#39441,#38285,#32352,.T.);
#51055=EDGE_CURVE('',#38278,#39443,#1277,.T.);
#51056=EDGE_CURVE('',#39442,#38282,#32353,.T.);
#51057=EDGE_CURVE('',#39483,#38253,#1278,.T.);
#51058=EDGE_CURVE('',#38248,#39482,#32354,.T.);
#51059=EDGE_CURVE('',#38247,#39481,#32355,.T.);
#51060=EDGE_CURVE('',#39472,#38255,#32356,.T.);
#51061=EDGE_CURVE('',#38244,#39480,#32357,.T.);
#51062=EDGE_CURVE('',#39473,#36993,#32358,.T.);
#51063=EDGE_CURVE('',#38243,#39479,#32359,.T.);
#51064=EDGE_CURVE('',#39474,#36992,#32360,.T.);
#51065=EDGE_CURVE('',#38241,#39478,#1279,.T.);
#51066=EDGE_CURVE('',#39457,#36991,#32361,.T.);
#51067=EDGE_CURVE('',#38236,#39477,#32362,.T.);
#51068=EDGE_CURVE('',#39458,#36990,#32363,.T.);
#51069=EDGE_CURVE('',#37222,#39476,#32364,.T.);
#51070=EDGE_CURVE('',#39463,#36989,#32365,.T.);
#51071=EDGE_CURVE('',#37223,#39475,#32366,.T.);
#51072=EDGE_CURVE('',#39464,#36988,#32367,.T.);
#51073=EDGE_CURVE('',#37224,#39456,#32368,.T.);
#51074=EDGE_CURVE('',#39465,#38274,#32369,.T.);
#51075=EDGE_CURVE('',#37225,#39459,#32370,.T.);
#51076=EDGE_CURVE('',#39466,#38270,#1280,.T.);
#51077=EDGE_CURVE('',#37226,#39462,#32371,.T.);
#51078=EDGE_CURVE('',#39467,#38269,#32372,.T.);
#51079=EDGE_CURVE('',#37227,#39461,#32373,.T.);
#51080=EDGE_CURVE('',#39468,#38266,#32374,.T.);
#51081=EDGE_CURVE('',#38257,#39460,#32375,.T.);
#51082=EDGE_CURVE('',#39469,#38265,#32376,.T.);
#51083=EDGE_CURVE('',#38258,#39471,#1281,.T.);
#51084=EDGE_CURVE('',#39470,#38262,#32377,.T.);
#51085=EDGE_CURVE('',#39511,#38233,#1282,.T.);
#51086=EDGE_CURVE('',#38228,#39510,#32378,.T.);
#51087=EDGE_CURVE('',#38227,#39509,#32379,.T.);
#51088=EDGE_CURVE('',#39500,#38235,#32380,.T.);
#51089=EDGE_CURVE('',#38224,#39508,#32381,.T.);
#51090=EDGE_CURVE('',#39501,#36999,#32382,.T.);
#51091=EDGE_CURVE('',#38223,#39507,#32383,.T.);
#51092=EDGE_CURVE('',#39502,#36998,#32384,.T.);
#51093=EDGE_CURVE('',#38221,#39506,#1283,.T.);
#51094=EDGE_CURVE('',#39485,#36997,#32385,.T.);
#51095=EDGE_CURVE('',#38216,#39505,#32386,.T.);
#51096=EDGE_CURVE('',#39486,#36996,#32387,.T.);
#51097=EDGE_CURVE('',#37216,#39504,#32388,.T.);
#51098=EDGE_CURVE('',#39491,#36995,#32389,.T.);
#51099=EDGE_CURVE('',#37217,#39503,#32390,.T.);
#51100=EDGE_CURVE('',#39492,#36994,#32391,.T.);
#51101=EDGE_CURVE('',#37218,#39484,#32392,.T.);
#51102=EDGE_CURVE('',#39493,#38254,#32393,.T.);
#51103=EDGE_CURVE('',#37219,#39487,#32394,.T.);
#51104=EDGE_CURVE('',#39494,#38250,#1284,.T.);
#51105=EDGE_CURVE('',#37220,#39490,#32395,.T.);
#51106=EDGE_CURVE('',#39495,#38249,#32396,.T.);
#51107=EDGE_CURVE('',#37221,#39489,#32397,.T.);
#51108=EDGE_CURVE('',#39496,#38246,#32398,.T.);
#51109=EDGE_CURVE('',#38237,#39488,#32399,.T.);
#51110=EDGE_CURVE('',#39497,#38245,#32400,.T.);
#51111=EDGE_CURVE('',#38238,#39499,#1285,.T.);
#51112=EDGE_CURVE('',#39498,#38242,#32401,.T.);
#51113=EDGE_CURVE('',#39539,#38213,#1286,.T.);
#51114=EDGE_CURVE('',#38208,#39538,#32402,.T.);
#51115=EDGE_CURVE('',#38207,#39537,#32403,.T.);
#51116=EDGE_CURVE('',#39528,#38215,#32404,.T.);
#51117=EDGE_CURVE('',#38204,#39536,#32405,.T.);
#51118=EDGE_CURVE('',#39529,#37005,#32406,.T.);
#51119=EDGE_CURVE('',#38203,#39535,#32407,.T.);
#51120=EDGE_CURVE('',#39530,#37004,#32408,.T.);
#51121=EDGE_CURVE('',#38201,#39534,#1287,.T.);
#51122=EDGE_CURVE('',#39513,#37003,#32409,.T.);
#51123=EDGE_CURVE('',#38196,#39533,#32410,.T.);
#51124=EDGE_CURVE('',#39514,#37002,#32411,.T.);
#51125=EDGE_CURVE('',#37210,#39532,#32412,.T.);
#51126=EDGE_CURVE('',#39519,#37001,#32413,.T.);
#51127=EDGE_CURVE('',#37211,#39531,#32414,.T.);
#51128=EDGE_CURVE('',#39520,#37000,#32415,.T.);
#51129=EDGE_CURVE('',#37212,#39512,#32416,.T.);
#51130=EDGE_CURVE('',#39521,#38234,#32417,.T.);
#51131=EDGE_CURVE('',#37213,#39515,#32418,.T.);
#51132=EDGE_CURVE('',#39522,#38230,#1288,.T.);
#51133=EDGE_CURVE('',#37214,#39518,#32419,.T.);
#51134=EDGE_CURVE('',#39523,#38229,#32420,.T.);
#51135=EDGE_CURVE('',#37215,#39517,#32421,.T.);
#51136=EDGE_CURVE('',#39524,#38226,#32422,.T.);
#51137=EDGE_CURVE('',#38217,#39516,#32423,.T.);
#51138=EDGE_CURVE('',#39525,#38225,#32424,.T.);
#51139=EDGE_CURVE('',#38218,#39527,#1289,.T.);
#51140=EDGE_CURVE('',#39526,#38222,#32425,.T.);
#51141=EDGE_CURVE('',#39567,#38193,#1290,.T.);
#51142=EDGE_CURVE('',#38188,#39566,#32426,.T.);
#51143=EDGE_CURVE('',#38187,#39565,#32427,.T.);
#51144=EDGE_CURVE('',#39556,#38195,#32428,.T.);
#51145=EDGE_CURVE('',#38184,#39564,#32429,.T.);
#51146=EDGE_CURVE('',#39557,#37011,#32430,.T.);
#51147=EDGE_CURVE('',#38183,#39563,#32431,.T.);
#51148=EDGE_CURVE('',#39558,#37010,#32432,.T.);
#51149=EDGE_CURVE('',#38181,#39562,#1291,.T.);
#51150=EDGE_CURVE('',#39541,#37009,#32433,.T.);
#51151=EDGE_CURVE('',#38176,#39561,#32434,.T.);
#51152=EDGE_CURVE('',#39542,#37008,#32435,.T.);
#51153=EDGE_CURVE('',#37204,#39560,#32436,.T.);
#51154=EDGE_CURVE('',#39547,#37007,#32437,.T.);
#51155=EDGE_CURVE('',#37205,#39559,#32438,.T.);
#51156=EDGE_CURVE('',#39548,#37006,#32439,.T.);
#51157=EDGE_CURVE('',#37206,#39540,#32440,.T.);
#51158=EDGE_CURVE('',#39549,#38214,#32441,.T.);
#51159=EDGE_CURVE('',#37207,#39543,#32442,.T.);
#51160=EDGE_CURVE('',#39550,#38210,#1292,.T.);
#51161=EDGE_CURVE('',#37208,#39546,#32443,.T.);
#51162=EDGE_CURVE('',#39551,#38209,#32444,.T.);
#51163=EDGE_CURVE('',#37209,#39545,#32445,.T.);
#51164=EDGE_CURVE('',#39552,#38206,#32446,.T.);
#51165=EDGE_CURVE('',#38197,#39544,#32447,.T.);
#51166=EDGE_CURVE('',#39553,#38205,#32448,.T.);
#51167=EDGE_CURVE('',#38198,#39555,#1293,.T.);
#51168=EDGE_CURVE('',#39554,#38202,#32449,.T.);
#51169=EDGE_CURVE('',#39595,#38173,#1294,.T.);
#51170=EDGE_CURVE('',#38168,#39594,#32450,.T.);
#51171=EDGE_CURVE('',#38167,#39593,#32451,.T.);
#51172=EDGE_CURVE('',#39584,#38175,#32452,.T.);
#51173=EDGE_CURVE('',#38164,#39592,#32453,.T.);
#51174=EDGE_CURVE('',#39585,#37017,#32454,.T.);
#51175=EDGE_CURVE('',#38163,#39591,#32455,.T.);
#51176=EDGE_CURVE('',#39586,#37016,#32456,.T.);
#51177=EDGE_CURVE('',#38161,#39590,#1295,.T.);
#51178=EDGE_CURVE('',#39569,#37015,#32457,.T.);
#51179=EDGE_CURVE('',#38156,#39589,#32458,.T.);
#51180=EDGE_CURVE('',#39570,#37014,#32459,.T.);
#51181=EDGE_CURVE('',#37198,#39588,#32460,.T.);
#51182=EDGE_CURVE('',#39575,#37013,#32461,.T.);
#51183=EDGE_CURVE('',#37199,#39587,#32462,.T.);
#51184=EDGE_CURVE('',#39576,#37012,#32463,.T.);
#51185=EDGE_CURVE('',#37200,#39568,#32464,.T.);
#51186=EDGE_CURVE('',#39577,#38194,#32465,.T.);
#51187=EDGE_CURVE('',#37201,#39571,#32466,.T.);
#51188=EDGE_CURVE('',#39578,#38190,#1296,.T.);
#51189=EDGE_CURVE('',#37202,#39574,#32467,.T.);
#51190=EDGE_CURVE('',#39579,#38189,#32468,.T.);
#51191=EDGE_CURVE('',#37203,#39573,#32469,.T.);
#51192=EDGE_CURVE('',#39580,#38186,#32470,.T.);
#51193=EDGE_CURVE('',#38177,#39572,#32471,.T.);
#51194=EDGE_CURVE('',#39581,#38185,#32472,.T.);
#51195=EDGE_CURVE('',#38178,#39583,#1297,.T.);
#51196=EDGE_CURVE('',#39582,#38182,#32473,.T.);
#51197=EDGE_CURVE('',#39619,#38153,#1298,.T.);
#51198=EDGE_CURVE('',#38148,#39618,#32474,.T.);
#51199=EDGE_CURVE('',#38147,#39617,#32475,.T.);
#51200=EDGE_CURVE('',#39608,#38155,#32476,.T.);
#51201=EDGE_CURVE('',#38144,#39616,#32477,.T.);
#51202=EDGE_CURVE('',#39609,#37021,#32478,.T.);
#51203=EDGE_CURVE('',#38143,#39615,#32479,.T.);
#51204=EDGE_CURVE('',#39610,#37020,#32480,.T.);
#51205=EDGE_CURVE('',#38141,#39614,#1299,.T.);
#51206=EDGE_CURVE('',#38136,#39613,#32481,.T.);
#51207=EDGE_CURVE('',#37551,#39612,#32482,.T.);
#51208=EDGE_CURVE('',#39599,#37019,#32483,.T.);
#51209=EDGE_CURVE('',#37552,#39611,#32484,.T.);
#51210=EDGE_CURVE('',#39600,#37018,#32485,.T.);
#51211=EDGE_CURVE('',#39601,#38174,#32486,.T.);
#51212=EDGE_CURVE('',#39602,#38170,#1300,.T.);
#51213=EDGE_CURVE('',#37196,#39598,#32487,.T.);
#51214=EDGE_CURVE('',#39603,#38169,#32488,.T.);
#51215=EDGE_CURVE('',#37197,#39597,#32489,.T.);
#51216=EDGE_CURVE('',#39604,#38166,#32490,.T.);
#51217=EDGE_CURVE('',#38157,#39596,#32491,.T.);
#51218=EDGE_CURVE('',#39605,#38165,#32492,.T.);
#51219=EDGE_CURVE('',#38158,#39607,#1301,.T.);
#51220=EDGE_CURVE('',#39606,#38162,#32493,.T.);
#51221=EDGE_CURVE('',#39647,#38133,#1302,.T.);
#51222=EDGE_CURVE('',#38128,#39646,#32494,.T.);
#51223=EDGE_CURVE('',#38127,#39645,#32495,.T.);
#51224=EDGE_CURVE('',#39636,#38135,#32496,.T.);
#51225=EDGE_CURVE('',#38124,#39644,#32497,.T.);
#51226=EDGE_CURVE('',#39637,#37027,#32498,.T.);
#51227=EDGE_CURVE('',#38123,#39643,#32499,.T.);
#51228=EDGE_CURVE('',#39638,#37026,#32500,.T.);
#51229=EDGE_CURVE('',#38121,#39642,#1303,.T.);
#51230=EDGE_CURVE('',#39621,#37025,#32501,.T.);
#51231=EDGE_CURVE('',#38116,#39641,#32502,.T.);
#51232=EDGE_CURVE('',#39622,#37024,#32503,.T.);
#51233=EDGE_CURVE('',#37545,#39640,#32504,.T.);
#51234=EDGE_CURVE('',#39627,#37023,#32505,.T.);
#51235=EDGE_CURVE('',#37546,#39639,#32506,.T.);
#51236=EDGE_CURVE('',#39628,#37022,#32507,.T.);
#51237=EDGE_CURVE('',#37547,#39620,#32508,.T.);
#51238=EDGE_CURVE('',#39629,#38154,#32509,.T.);
#51239=EDGE_CURVE('',#37548,#39623,#32510,.T.);
#51240=EDGE_CURVE('',#39630,#38150,#1304,.T.);
#51241=EDGE_CURVE('',#37549,#39626,#32511,.T.);
#51242=EDGE_CURVE('',#39631,#38149,#32512,.T.);
#51243=EDGE_CURVE('',#37550,#39625,#32513,.T.);
#51244=EDGE_CURVE('',#39632,#38146,#32514,.T.);
#51245=EDGE_CURVE('',#38137,#39624,#32515,.T.);
#51246=EDGE_CURVE('',#39633,#38145,#32516,.T.);
#51247=EDGE_CURVE('',#38138,#39635,#1305,.T.);
#51248=EDGE_CURVE('',#39634,#38142,#32517,.T.);
#51249=EDGE_CURVE('',#39675,#38113,#1306,.T.);
#51250=EDGE_CURVE('',#38108,#39674,#32518,.T.);
#51251=EDGE_CURVE('',#38107,#39673,#32519,.T.);
#51252=EDGE_CURVE('',#39664,#38115,#32520,.T.);
#51253=EDGE_CURVE('',#38104,#39672,#32521,.T.);
#51254=EDGE_CURVE('',#39665,#37033,#32522,.T.);
#51255=EDGE_CURVE('',#38103,#39671,#32523,.T.);
#51256=EDGE_CURVE('',#39666,#37032,#32524,.T.);
#51257=EDGE_CURVE('',#38101,#39670,#1307,.T.);
#51258=EDGE_CURVE('',#39649,#37031,#32525,.T.);
#51259=EDGE_CURVE('',#38096,#39669,#32526,.T.);
#51260=EDGE_CURVE('',#39650,#37030,#32527,.T.);
#51261=EDGE_CURVE('',#37539,#39668,#32528,.T.);
#51262=EDGE_CURVE('',#39655,#37029,#32529,.T.);
#51263=EDGE_CURVE('',#37540,#39667,#32530,.T.);
#51264=EDGE_CURVE('',#39656,#37028,#32531,.T.);
#51265=EDGE_CURVE('',#37541,#39648,#32532,.T.);
#51266=EDGE_CURVE('',#39657,#38134,#32533,.T.);
#51267=EDGE_CURVE('',#37542,#39651,#32534,.T.);
#51268=EDGE_CURVE('',#39658,#38130,#1308,.T.);
#51269=EDGE_CURVE('',#37543,#39654,#32535,.T.);
#51270=EDGE_CURVE('',#39659,#38129,#32536,.T.);
#51271=EDGE_CURVE('',#37544,#39653,#32537,.T.);
#51272=EDGE_CURVE('',#39660,#38126,#32538,.T.);
#51273=EDGE_CURVE('',#38117,#39652,#32539,.T.);
#51274=EDGE_CURVE('',#39661,#38125,#32540,.T.);
#51275=EDGE_CURVE('',#38118,#39663,#1309,.T.);
#51276=EDGE_CURVE('',#39662,#38122,#32541,.T.);
#51277=EDGE_CURVE('',#39703,#38093,#1310,.T.);
#51278=EDGE_CURVE('',#38088,#39702,#32542,.T.);
#51279=EDGE_CURVE('',#38087,#39701,#32543,.T.);
#51280=EDGE_CURVE('',#39692,#38095,#32544,.T.);
#51281=EDGE_CURVE('',#38084,#39700,#32545,.T.);
#51282=EDGE_CURVE('',#39693,#37039,#32546,.T.);
#51283=EDGE_CURVE('',#38083,#39699,#32547,.T.);
#51284=EDGE_CURVE('',#39694,#37038,#32548,.T.);
#51285=EDGE_CURVE('',#38081,#39698,#1311,.T.);
#51286=EDGE_CURVE('',#39677,#37037,#32549,.T.);
#51287=EDGE_CURVE('',#38076,#39697,#32550,.T.);
#51288=EDGE_CURVE('',#39678,#37036,#32551,.T.);
#51289=EDGE_CURVE('',#37533,#39696,#32552,.T.);
#51290=EDGE_CURVE('',#39683,#37035,#32553,.T.);
#51291=EDGE_CURVE('',#37534,#39695,#32554,.T.);
#51292=EDGE_CURVE('',#39684,#37034,#32555,.T.);
#51293=EDGE_CURVE('',#37535,#39676,#32556,.T.);
#51294=EDGE_CURVE('',#39685,#38114,#32557,.T.);
#51295=EDGE_CURVE('',#37536,#39679,#32558,.T.);
#51296=EDGE_CURVE('',#39686,#38110,#1312,.T.);
#51297=EDGE_CURVE('',#37537,#39682,#32559,.T.);
#51298=EDGE_CURVE('',#39687,#38109,#32560,.T.);
#51299=EDGE_CURVE('',#37538,#39681,#32561,.T.);
#51300=EDGE_CURVE('',#39688,#38106,#32562,.T.);
#51301=EDGE_CURVE('',#38097,#39680,#32563,.T.);
#51302=EDGE_CURVE('',#39689,#38105,#32564,.T.);
#51303=EDGE_CURVE('',#38098,#39691,#1313,.T.);
#51304=EDGE_CURVE('',#39690,#38102,#32565,.T.);
#51305=EDGE_CURVE('',#39731,#38073,#1314,.T.);
#51306=EDGE_CURVE('',#38068,#39730,#32566,.T.);
#51307=EDGE_CURVE('',#38067,#39729,#32567,.T.);
#51308=EDGE_CURVE('',#39720,#38075,#32568,.T.);
#51309=EDGE_CURVE('',#38064,#39728,#32569,.T.);
#51310=EDGE_CURVE('',#39721,#37045,#32570,.T.);
#51311=EDGE_CURVE('',#38063,#39727,#32571,.T.);
#51312=EDGE_CURVE('',#39722,#37044,#32572,.T.);
#51313=EDGE_CURVE('',#38061,#39726,#1315,.T.);
#51314=EDGE_CURVE('',#39705,#37043,#32573,.T.);
#51315=EDGE_CURVE('',#38056,#39725,#32574,.T.);
#51316=EDGE_CURVE('',#39706,#37042,#32575,.T.);
#51317=EDGE_CURVE('',#37527,#39724,#32576,.T.);
#51318=EDGE_CURVE('',#39711,#37041,#32577,.T.);
#51319=EDGE_CURVE('',#37528,#39723,#32578,.T.);
#51320=EDGE_CURVE('',#39712,#37040,#32579,.T.);
#51321=EDGE_CURVE('',#37529,#39704,#32580,.T.);
#51322=EDGE_CURVE('',#39713,#38094,#32581,.T.);
#51323=EDGE_CURVE('',#37530,#39707,#32582,.T.);
#51324=EDGE_CURVE('',#39714,#38090,#1316,.T.);
#51325=EDGE_CURVE('',#37531,#39710,#32583,.T.);
#51326=EDGE_CURVE('',#39715,#38089,#32584,.T.);
#51327=EDGE_CURVE('',#37532,#39709,#32585,.T.);
#51328=EDGE_CURVE('',#39716,#38086,#32586,.T.);
#51329=EDGE_CURVE('',#38077,#39708,#32587,.T.);
#51330=EDGE_CURVE('',#39717,#38085,#32588,.T.);
#51331=EDGE_CURVE('',#38078,#39719,#1317,.T.);
#51332=EDGE_CURVE('',#39718,#38082,#32589,.T.);
#51333=EDGE_CURVE('',#39759,#38053,#1318,.T.);
#51334=EDGE_CURVE('',#38048,#39758,#32590,.T.);
#51335=EDGE_CURVE('',#38047,#39757,#32591,.T.);
#51336=EDGE_CURVE('',#39748,#38055,#32592,.T.);
#51337=EDGE_CURVE('',#38044,#39756,#32593,.T.);
#51338=EDGE_CURVE('',#39749,#37051,#32594,.T.);
#51339=EDGE_CURVE('',#38043,#39755,#32595,.T.);
#51340=EDGE_CURVE('',#39750,#37050,#32596,.T.);
#51341=EDGE_CURVE('',#38041,#39754,#1319,.T.);
#51342=EDGE_CURVE('',#39733,#37049,#32597,.T.);
#51343=EDGE_CURVE('',#38036,#39753,#32598,.T.);
#51344=EDGE_CURVE('',#39734,#37048,#32599,.T.);
#51345=EDGE_CURVE('',#37521,#39752,#32600,.T.);
#51346=EDGE_CURVE('',#39739,#37047,#32601,.T.);
#51347=EDGE_CURVE('',#37522,#39751,#32602,.T.);
#51348=EDGE_CURVE('',#39740,#37046,#32603,.T.);
#51349=EDGE_CURVE('',#37523,#39732,#32604,.T.);
#51350=EDGE_CURVE('',#39741,#38074,#32605,.T.);
#51351=EDGE_CURVE('',#37524,#39735,#32606,.T.);
#51352=EDGE_CURVE('',#39742,#38070,#1320,.T.);
#51353=EDGE_CURVE('',#37525,#39738,#32607,.T.);
#51354=EDGE_CURVE('',#39743,#38069,#32608,.T.);
#51355=EDGE_CURVE('',#37526,#39737,#32609,.T.);
#51356=EDGE_CURVE('',#39744,#38066,#32610,.T.);
#51357=EDGE_CURVE('',#38057,#39736,#32611,.T.);
#51358=EDGE_CURVE('',#39745,#38065,#32612,.T.);
#51359=EDGE_CURVE('',#38058,#39747,#1321,.T.);
#51360=EDGE_CURVE('',#39746,#38062,#32613,.T.);
#51361=EDGE_CURVE('',#39787,#38033,#1322,.T.);
#51362=EDGE_CURVE('',#38028,#39786,#32614,.T.);
#51363=EDGE_CURVE('',#38027,#39785,#32615,.T.);
#51364=EDGE_CURVE('',#39776,#38035,#32616,.T.);
#51365=EDGE_CURVE('',#38024,#39784,#32617,.T.);
#51366=EDGE_CURVE('',#39777,#37057,#32618,.T.);
#51367=EDGE_CURVE('',#38023,#39783,#32619,.T.);
#51368=EDGE_CURVE('',#39778,#37056,#32620,.T.);
#51369=EDGE_CURVE('',#38021,#39782,#1323,.T.);
#51370=EDGE_CURVE('',#39761,#37055,#32621,.T.);
#51371=EDGE_CURVE('',#38016,#39781,#32622,.T.);
#51372=EDGE_CURVE('',#39762,#37054,#32623,.T.);
#51373=EDGE_CURVE('',#37515,#39780,#32624,.T.);
#51374=EDGE_CURVE('',#39767,#37053,#32625,.T.);
#51375=EDGE_CURVE('',#37516,#39779,#32626,.T.);
#51376=EDGE_CURVE('',#39768,#37052,#32627,.T.);
#51377=EDGE_CURVE('',#37517,#39760,#32628,.T.);
#51378=EDGE_CURVE('',#39769,#38054,#32629,.T.);
#51379=EDGE_CURVE('',#37518,#39763,#32630,.T.);
#51380=EDGE_CURVE('',#39770,#38050,#1324,.T.);
#51381=EDGE_CURVE('',#37519,#39766,#32631,.T.);
#51382=EDGE_CURVE('',#39771,#38049,#32632,.T.);
#51383=EDGE_CURVE('',#37520,#39765,#32633,.T.);
#51384=EDGE_CURVE('',#39772,#38046,#32634,.T.);
#51385=EDGE_CURVE('',#38037,#39764,#32635,.T.);
#51386=EDGE_CURVE('',#39773,#38045,#32636,.T.);
#51387=EDGE_CURVE('',#38038,#39775,#1325,.T.);
#51388=EDGE_CURVE('',#39774,#38042,#32637,.T.);
#51389=EDGE_CURVE('',#39815,#38013,#1326,.T.);
#51390=EDGE_CURVE('',#38008,#39814,#32638,.T.);
#51391=EDGE_CURVE('',#38007,#39813,#32639,.T.);
#51392=EDGE_CURVE('',#39804,#38015,#32640,.T.);
#51393=EDGE_CURVE('',#38004,#39812,#32641,.T.);
#51394=EDGE_CURVE('',#39805,#37063,#32642,.T.);
#51395=EDGE_CURVE('',#38003,#39811,#32643,.T.);
#51396=EDGE_CURVE('',#39806,#37062,#32644,.T.);
#51397=EDGE_CURVE('',#38001,#39810,#1327,.T.);
#51398=EDGE_CURVE('',#39789,#37061,#32645,.T.);
#51399=EDGE_CURVE('',#37996,#39809,#32646,.T.);
#51400=EDGE_CURVE('',#39790,#37060,#32647,.T.);
#51401=EDGE_CURVE('',#37509,#39808,#32648,.T.);
#51402=EDGE_CURVE('',#39795,#37059,#32649,.T.);
#51403=EDGE_CURVE('',#37510,#39807,#32650,.T.);
#51404=EDGE_CURVE('',#39796,#37058,#32651,.T.);
#51405=EDGE_CURVE('',#37511,#39788,#32652,.T.);
#51406=EDGE_CURVE('',#39797,#38034,#32653,.T.);
#51407=EDGE_CURVE('',#37512,#39791,#32654,.T.);
#51408=EDGE_CURVE('',#39798,#38030,#1328,.T.);
#51409=EDGE_CURVE('',#37513,#39794,#32655,.T.);
#51410=EDGE_CURVE('',#39799,#38029,#32656,.T.);
#51411=EDGE_CURVE('',#37514,#39793,#32657,.T.);
#51412=EDGE_CURVE('',#39800,#38026,#32658,.T.);
#51413=EDGE_CURVE('',#38017,#39792,#32659,.T.);
#51414=EDGE_CURVE('',#39801,#38025,#32660,.T.);
#51415=EDGE_CURVE('',#38018,#39803,#1329,.T.);
#51416=EDGE_CURVE('',#39802,#38022,#32661,.T.);
#51417=EDGE_CURVE('',#39843,#37993,#1330,.T.);
#51418=EDGE_CURVE('',#37988,#39842,#32662,.T.);
#51419=EDGE_CURVE('',#37987,#39841,#32663,.T.);
#51420=EDGE_CURVE('',#39832,#37995,#32664,.T.);
#51421=EDGE_CURVE('',#37984,#39840,#32665,.T.);
#51422=EDGE_CURVE('',#39833,#37069,#32666,.T.);
#51423=EDGE_CURVE('',#37983,#39839,#32667,.T.);
#51424=EDGE_CURVE('',#39834,#37068,#32668,.T.);
#51425=EDGE_CURVE('',#37981,#39838,#1331,.T.);
#51426=EDGE_CURVE('',#39817,#37067,#32669,.T.);
#51427=EDGE_CURVE('',#37976,#39837,#32670,.T.);
#51428=EDGE_CURVE('',#39818,#37066,#32671,.T.);
#51429=EDGE_CURVE('',#37503,#39836,#32672,.T.);
#51430=EDGE_CURVE('',#39823,#37065,#32673,.T.);
#51431=EDGE_CURVE('',#37504,#39835,#32674,.T.);
#51432=EDGE_CURVE('',#39824,#37064,#32675,.T.);
#51433=EDGE_CURVE('',#37505,#39816,#32676,.T.);
#51434=EDGE_CURVE('',#39825,#38014,#32677,.T.);
#51435=EDGE_CURVE('',#37506,#39819,#32678,.T.);
#51436=EDGE_CURVE('',#39826,#38010,#1332,.T.);
#51437=EDGE_CURVE('',#37507,#39822,#32679,.T.);
#51438=EDGE_CURVE('',#39827,#38009,#32680,.T.);
#51439=EDGE_CURVE('',#37508,#39821,#32681,.T.);
#51440=EDGE_CURVE('',#39828,#38006,#32682,.T.);
#51441=EDGE_CURVE('',#37997,#39820,#32683,.T.);
#51442=EDGE_CURVE('',#39829,#38005,#32684,.T.);
#51443=EDGE_CURVE('',#37998,#39831,#1333,.T.);
#51444=EDGE_CURVE('',#39830,#38002,#32685,.T.);
#51445=EDGE_CURVE('',#39871,#37973,#1334,.T.);
#51446=EDGE_CURVE('',#37968,#39870,#32686,.T.);
#51447=EDGE_CURVE('',#37967,#39869,#32687,.T.);
#51448=EDGE_CURVE('',#39860,#37975,#32688,.T.);
#51449=EDGE_CURVE('',#37964,#39868,#32689,.T.);
#51450=EDGE_CURVE('',#39861,#37075,#32690,.T.);
#51451=EDGE_CURVE('',#37963,#39867,#32691,.T.);
#51452=EDGE_CURVE('',#39862,#37074,#32692,.T.);
#51453=EDGE_CURVE('',#37961,#39866,#1335,.T.);
#51454=EDGE_CURVE('',#39845,#37073,#32693,.T.);
#51455=EDGE_CURVE('',#37956,#39865,#32694,.T.);
#51456=EDGE_CURVE('',#39846,#37072,#32695,.T.);
#51457=EDGE_CURVE('',#37497,#39864,#32696,.T.);
#51458=EDGE_CURVE('',#39851,#37071,#32697,.T.);
#51459=EDGE_CURVE('',#37498,#39863,#32698,.T.);
#51460=EDGE_CURVE('',#39852,#37070,#32699,.T.);
#51461=EDGE_CURVE('',#37499,#39844,#32700,.T.);
#51462=EDGE_CURVE('',#39853,#37994,#32701,.T.);
#51463=EDGE_CURVE('',#37500,#39847,#32702,.T.);
#51464=EDGE_CURVE('',#39854,#37990,#1336,.T.);
#51465=EDGE_CURVE('',#37501,#39850,#32703,.T.);
#51466=EDGE_CURVE('',#39855,#37989,#32704,.T.);
#51467=EDGE_CURVE('',#37502,#39849,#32705,.T.);
#51468=EDGE_CURVE('',#39856,#37986,#32706,.T.);
#51469=EDGE_CURVE('',#37977,#39848,#32707,.T.);
#51470=EDGE_CURVE('',#39857,#37985,#32708,.T.);
#51471=EDGE_CURVE('',#37978,#39859,#1337,.T.);
#51472=EDGE_CURVE('',#39858,#37982,#32709,.T.);
#51473=EDGE_CURVE('',#39899,#37953,#1338,.T.);
#51474=EDGE_CURVE('',#37948,#39898,#32710,.T.);
#51475=EDGE_CURVE('',#37947,#39897,#32711,.T.);
#51476=EDGE_CURVE('',#39888,#37955,#32712,.T.);
#51477=EDGE_CURVE('',#37944,#39896,#32713,.T.);
#51478=EDGE_CURVE('',#39889,#37081,#32714,.T.);
#51479=EDGE_CURVE('',#37943,#39895,#32715,.T.);
#51480=EDGE_CURVE('',#39890,#37080,#32716,.T.);
#51481=EDGE_CURVE('',#37941,#39894,#1339,.T.);
#51482=EDGE_CURVE('',#39873,#37079,#32717,.T.);
#51483=EDGE_CURVE('',#37936,#39893,#32718,.T.);
#51484=EDGE_CURVE('',#39874,#37078,#32719,.T.);
#51485=EDGE_CURVE('',#37491,#39892,#32720,.T.);
#51486=EDGE_CURVE('',#39879,#37077,#32721,.T.);
#51487=EDGE_CURVE('',#37492,#39891,#32722,.T.);
#51488=EDGE_CURVE('',#39880,#37076,#32723,.T.);
#51489=EDGE_CURVE('',#37493,#39872,#32724,.T.);
#51490=EDGE_CURVE('',#39881,#37974,#32725,.T.);
#51491=EDGE_CURVE('',#37494,#39875,#32726,.T.);
#51492=EDGE_CURVE('',#39882,#37970,#1340,.T.);
#51493=EDGE_CURVE('',#37495,#39878,#32727,.T.);
#51494=EDGE_CURVE('',#39883,#37969,#32728,.T.);
#51495=EDGE_CURVE('',#37496,#39877,#32729,.T.);
#51496=EDGE_CURVE('',#39884,#37966,#32730,.T.);
#51497=EDGE_CURVE('',#37957,#39876,#32731,.T.);
#51498=EDGE_CURVE('',#39885,#37965,#32732,.T.);
#51499=EDGE_CURVE('',#37958,#39887,#1341,.T.);
#51500=EDGE_CURVE('',#39886,#37962,#32733,.T.);
#51501=EDGE_CURVE('',#39927,#37933,#1342,.T.);
#51502=EDGE_CURVE('',#37928,#39926,#32734,.T.);
#51503=EDGE_CURVE('',#37927,#39925,#32735,.T.);
#51504=EDGE_CURVE('',#39916,#37935,#32736,.T.);
#51505=EDGE_CURVE('',#37924,#39924,#32737,.T.);
#51506=EDGE_CURVE('',#39917,#37087,#32738,.T.);
#51507=EDGE_CURVE('',#37923,#39923,#32739,.T.);
#51508=EDGE_CURVE('',#39918,#37086,#32740,.T.);
#51509=EDGE_CURVE('',#37921,#39922,#1343,.T.);
#51510=EDGE_CURVE('',#39901,#37085,#32741,.T.);
#51511=EDGE_CURVE('',#37916,#39921,#32742,.T.);
#51512=EDGE_CURVE('',#39902,#37084,#32743,.T.);
#51513=EDGE_CURVE('',#37485,#39920,#32744,.T.);
#51514=EDGE_CURVE('',#39907,#37083,#32745,.T.);
#51515=EDGE_CURVE('',#37486,#39919,#32746,.T.);
#51516=EDGE_CURVE('',#39908,#37082,#32747,.T.);
#51517=EDGE_CURVE('',#37487,#39900,#32748,.T.);
#51518=EDGE_CURVE('',#39909,#37954,#32749,.T.);
#51519=EDGE_CURVE('',#37488,#39903,#32750,.T.);
#51520=EDGE_CURVE('',#39910,#37950,#1344,.T.);
#51521=EDGE_CURVE('',#37489,#39906,#32751,.T.);
#51522=EDGE_CURVE('',#39911,#37949,#32752,.T.);
#51523=EDGE_CURVE('',#37490,#39905,#32753,.T.);
#51524=EDGE_CURVE('',#39912,#37946,#32754,.T.);
#51525=EDGE_CURVE('',#37937,#39904,#32755,.T.);
#51526=EDGE_CURVE('',#39913,#37945,#32756,.T.);
#51527=EDGE_CURVE('',#37938,#39915,#1345,.T.);
#51528=EDGE_CURVE('',#39914,#37942,#32757,.T.);
#51529=EDGE_CURVE('',#39955,#37913,#1346,.T.);
#51530=EDGE_CURVE('',#37908,#39954,#32758,.T.);
#51531=EDGE_CURVE('',#37907,#39953,#32759,.T.);
#51532=EDGE_CURVE('',#39944,#37915,#32760,.T.);
#51533=EDGE_CURVE('',#37904,#39952,#32761,.T.);
#51534=EDGE_CURVE('',#39945,#37093,#32762,.T.);
#51535=EDGE_CURVE('',#37903,#39951,#32763,.T.);
#51536=EDGE_CURVE('',#39946,#37092,#32764,.T.);
#51537=EDGE_CURVE('',#37901,#39950,#1347,.T.);
#51538=EDGE_CURVE('',#39929,#37091,#32765,.T.);
#51539=EDGE_CURVE('',#37896,#39949,#32766,.T.);
#51540=EDGE_CURVE('',#39930,#37090,#32767,.T.);
#51541=EDGE_CURVE('',#37479,#39948,#32768,.T.);
#51542=EDGE_CURVE('',#39935,#37089,#32769,.T.);
#51543=EDGE_CURVE('',#37480,#39947,#32770,.T.);
#51544=EDGE_CURVE('',#39936,#37088,#32771,.T.);
#51545=EDGE_CURVE('',#37481,#39928,#32772,.T.);
#51546=EDGE_CURVE('',#39937,#37934,#32773,.T.);
#51547=EDGE_CURVE('',#37482,#39931,#32774,.T.);
#51548=EDGE_CURVE('',#39938,#37930,#1348,.T.);
#51549=EDGE_CURVE('',#37483,#39934,#32775,.T.);
#51550=EDGE_CURVE('',#39939,#37929,#32776,.T.);
#51551=EDGE_CURVE('',#37484,#39933,#32777,.T.);
#51552=EDGE_CURVE('',#39940,#37926,#32778,.T.);
#51553=EDGE_CURVE('',#37917,#39932,#32779,.T.);
#51554=EDGE_CURVE('',#39941,#37925,#32780,.T.);
#51555=EDGE_CURVE('',#37918,#39943,#1349,.T.);
#51556=EDGE_CURVE('',#39942,#37922,#32781,.T.);
#51557=EDGE_CURVE('',#39983,#37893,#1350,.T.);
#51558=EDGE_CURVE('',#37888,#39982,#32782,.T.);
#51559=EDGE_CURVE('',#37887,#39981,#32783,.T.);
#51560=EDGE_CURVE('',#39972,#37895,#32784,.T.);
#51561=EDGE_CURVE('',#37884,#39980,#32785,.T.);
#51562=EDGE_CURVE('',#39973,#37099,#32786,.T.);
#51563=EDGE_CURVE('',#37883,#39979,#32787,.T.);
#51564=EDGE_CURVE('',#39974,#37098,#32788,.T.);
#51565=EDGE_CURVE('',#37881,#39978,#1351,.T.);
#51566=EDGE_CURVE('',#39957,#37097,#32789,.T.);
#51567=EDGE_CURVE('',#37876,#39977,#32790,.T.);
#51568=EDGE_CURVE('',#39958,#37096,#32791,.T.);
#51569=EDGE_CURVE('',#37473,#39976,#32792,.T.);
#51570=EDGE_CURVE('',#39963,#37095,#32793,.T.);
#51571=EDGE_CURVE('',#37474,#39975,#32794,.T.);
#51572=EDGE_CURVE('',#39964,#37094,#32795,.T.);
#51573=EDGE_CURVE('',#37475,#39956,#32796,.T.);
#51574=EDGE_CURVE('',#39965,#37914,#32797,.T.);
#51575=EDGE_CURVE('',#37476,#39959,#32798,.T.);
#51576=EDGE_CURVE('',#39966,#37910,#1352,.T.);
#51577=EDGE_CURVE('',#37477,#39962,#32799,.T.);
#51578=EDGE_CURVE('',#39967,#37909,#32800,.T.);
#51579=EDGE_CURVE('',#37478,#39961,#32801,.T.);
#51580=EDGE_CURVE('',#39968,#37906,#32802,.T.);
#51581=EDGE_CURVE('',#37897,#39960,#32803,.T.);
#51582=EDGE_CURVE('',#39969,#37905,#32804,.T.);
#51583=EDGE_CURVE('',#37898,#39971,#1353,.T.);
#51584=EDGE_CURVE('',#39970,#37902,#32805,.T.);
#51585=EDGE_CURVE('',#40011,#37873,#1354,.T.);
#51586=EDGE_CURVE('',#37868,#40010,#32806,.T.);
#51587=EDGE_CURVE('',#37867,#40009,#32807,.T.);
#51588=EDGE_CURVE('',#40000,#37875,#32808,.T.);
#51589=EDGE_CURVE('',#37864,#40008,#32809,.T.);
#51590=EDGE_CURVE('',#40001,#37105,#32810,.T.);
#51591=EDGE_CURVE('',#37863,#40007,#32811,.T.);
#51592=EDGE_CURVE('',#40002,#37104,#32812,.T.);
#51593=EDGE_CURVE('',#37861,#40006,#1355,.T.);
#51594=EDGE_CURVE('',#39985,#37103,#32813,.T.);
#51595=EDGE_CURVE('',#37856,#40005,#32814,.T.);
#51596=EDGE_CURVE('',#39986,#37102,#32815,.T.);
#51597=EDGE_CURVE('',#37467,#40004,#32816,.T.);
#51598=EDGE_CURVE('',#39991,#37101,#32817,.T.);
#51599=EDGE_CURVE('',#37468,#40003,#32818,.T.);
#51600=EDGE_CURVE('',#39992,#37100,#32819,.T.);
#51601=EDGE_CURVE('',#37469,#39984,#32820,.T.);
#51602=EDGE_CURVE('',#39993,#37894,#32821,.T.);
#51603=EDGE_CURVE('',#37470,#39987,#32822,.T.);
#51604=EDGE_CURVE('',#39994,#37890,#1356,.T.);
#51605=EDGE_CURVE('',#37471,#39990,#32823,.T.);
#51606=EDGE_CURVE('',#39995,#37889,#32824,.T.);
#51607=EDGE_CURVE('',#37472,#39989,#32825,.T.);
#51608=EDGE_CURVE('',#39996,#37886,#32826,.T.);
#51609=EDGE_CURVE('',#37877,#39988,#32827,.T.);
#51610=EDGE_CURVE('',#39997,#37885,#32828,.T.);
#51611=EDGE_CURVE('',#37878,#39999,#1357,.T.);
#51612=EDGE_CURVE('',#39998,#37882,#32829,.T.);
#51613=EDGE_CURVE('',#40035,#37853,#1358,.T.);
#51614=EDGE_CURVE('',#37848,#40034,#32830,.T.);
#51615=EDGE_CURVE('',#37847,#40033,#32831,.T.);
#51616=EDGE_CURVE('',#40024,#37855,#32832,.T.);
#51617=EDGE_CURVE('',#37844,#40032,#32833,.T.);
#51618=EDGE_CURVE('',#40025,#37109,#32834,.T.);
#51619=EDGE_CURVE('',#37843,#40031,#32835,.T.);
#51620=EDGE_CURVE('',#40026,#37108,#32836,.T.);
#51621=EDGE_CURVE('',#37841,#40030,#1359,.T.);
#51622=EDGE_CURVE('',#37836,#40029,#32837,.T.);
#51623=EDGE_CURVE('',#37463,#40028,#32838,.T.);
#51624=EDGE_CURVE('',#40015,#37107,#32839,.T.);
#51625=EDGE_CURVE('',#37464,#40027,#32840,.T.);
#51626=EDGE_CURVE('',#40016,#37106,#32841,.T.);
#51627=EDGE_CURVE('',#40017,#37874,#32842,.T.);
#51628=EDGE_CURVE('',#40018,#37870,#1360,.T.);
#51629=EDGE_CURVE('',#37465,#40014,#32843,.T.);
#51630=EDGE_CURVE('',#40019,#37869,#32844,.T.);
#51631=EDGE_CURVE('',#37466,#40013,#32845,.T.);
#51632=EDGE_CURVE('',#40020,#37866,#32846,.T.);
#51633=EDGE_CURVE('',#37857,#40012,#32847,.T.);
#51634=EDGE_CURVE('',#40021,#37865,#32848,.T.);
#51635=EDGE_CURVE('',#37858,#40023,#1361,.T.);
#51636=EDGE_CURVE('',#40022,#37862,#32849,.T.);
#51637=EDGE_CURVE('',#40063,#37833,#1362,.T.);
#51638=EDGE_CURVE('',#37828,#40062,#32850,.T.);
#51639=EDGE_CURVE('',#37827,#40061,#32851,.T.);
#51640=EDGE_CURVE('',#40052,#37835,#32852,.T.);
#51641=EDGE_CURVE('',#37824,#40060,#32853,.T.);
#51642=EDGE_CURVE('',#40053,#37115,#32854,.T.);
#51643=EDGE_CURVE('',#37823,#40059,#32855,.T.);
#51644=EDGE_CURVE('',#40054,#37114,#32856,.T.);
#51645=EDGE_CURVE('',#37821,#40058,#1363,.T.);
#51646=EDGE_CURVE('',#40037,#37113,#32857,.T.);
#51647=EDGE_CURVE('',#37816,#40057,#32858,.T.);
#51648=EDGE_CURVE('',#40038,#37112,#32859,.T.);
#51649=EDGE_CURVE('',#37457,#40056,#32860,.T.);
#51650=EDGE_CURVE('',#40043,#37111,#32861,.T.);
#51651=EDGE_CURVE('',#37458,#40055,#32862,.T.);
#51652=EDGE_CURVE('',#40044,#37110,#32863,.T.);
#51653=EDGE_CURVE('',#37459,#40036,#32864,.T.);
#51654=EDGE_CURVE('',#40045,#37854,#32865,.T.);
#51655=EDGE_CURVE('',#37460,#40039,#32866,.T.);
#51656=EDGE_CURVE('',#40046,#37850,#1364,.T.);
#51657=EDGE_CURVE('',#37461,#40042,#32867,.T.);
#51658=EDGE_CURVE('',#40047,#37849,#32868,.T.);
#51659=EDGE_CURVE('',#37462,#40041,#32869,.T.);
#51660=EDGE_CURVE('',#40048,#37846,#32870,.T.);
#51661=EDGE_CURVE('',#37837,#40040,#32871,.T.);
#51662=EDGE_CURVE('',#40049,#37845,#32872,.T.);
#51663=EDGE_CURVE('',#37838,#40051,#1365,.T.);
#51664=EDGE_CURVE('',#40050,#37842,#32873,.T.);
#51665=EDGE_CURVE('',#40091,#37813,#1366,.T.);
#51666=EDGE_CURVE('',#37808,#40090,#32874,.T.);
#51667=EDGE_CURVE('',#37807,#40089,#32875,.T.);
#51668=EDGE_CURVE('',#40080,#37815,#32876,.T.);
#51669=EDGE_CURVE('',#37804,#40088,#32877,.T.);
#51670=EDGE_CURVE('',#40081,#37121,#32878,.T.);
#51671=EDGE_CURVE('',#37803,#40087,#32879,.T.);
#51672=EDGE_CURVE('',#40082,#37120,#32880,.T.);
#51673=EDGE_CURVE('',#37801,#40086,#1367,.T.);
#51674=EDGE_CURVE('',#40065,#37119,#32881,.T.);
#51675=EDGE_CURVE('',#37796,#40085,#32882,.T.);
#51676=EDGE_CURVE('',#40066,#37118,#32883,.T.);
#51677=EDGE_CURVE('',#37451,#40084,#32884,.T.);
#51678=EDGE_CURVE('',#40071,#37117,#32885,.T.);
#51679=EDGE_CURVE('',#37452,#40083,#32886,.T.);
#51680=EDGE_CURVE('',#40072,#37116,#32887,.T.);
#51681=EDGE_CURVE('',#37453,#40064,#32888,.T.);
#51682=EDGE_CURVE('',#40073,#37834,#32889,.T.);
#51683=EDGE_CURVE('',#37454,#40067,#32890,.T.);
#51684=EDGE_CURVE('',#40074,#37830,#1368,.T.);
#51685=EDGE_CURVE('',#37455,#40070,#32891,.T.);
#51686=EDGE_CURVE('',#40075,#37829,#32892,.T.);
#51687=EDGE_CURVE('',#37456,#40069,#32893,.T.);
#51688=EDGE_CURVE('',#40076,#37826,#32894,.T.);
#51689=EDGE_CURVE('',#37817,#40068,#32895,.T.);
#51690=EDGE_CURVE('',#40077,#37825,#32896,.T.);
#51691=EDGE_CURVE('',#37818,#40079,#1369,.T.);
#51692=EDGE_CURVE('',#40078,#37822,#32897,.T.);
#51693=EDGE_CURVE('',#40119,#37793,#1370,.T.);
#51694=EDGE_CURVE('',#37788,#40118,#32898,.T.);
#51695=EDGE_CURVE('',#37787,#40117,#32899,.T.);
#51696=EDGE_CURVE('',#40108,#37795,#32900,.T.);
#51697=EDGE_CURVE('',#37784,#40116,#32901,.T.);
#51698=EDGE_CURVE('',#40109,#37127,#32902,.T.);
#51699=EDGE_CURVE('',#37783,#40115,#32903,.T.);
#51700=EDGE_CURVE('',#40110,#37126,#32904,.T.);
#51701=EDGE_CURVE('',#37781,#40114,#1371,.T.);
#51702=EDGE_CURVE('',#40093,#37125,#32905,.T.);
#51703=EDGE_CURVE('',#37776,#40113,#32906,.T.);
#51704=EDGE_CURVE('',#40094,#37124,#32907,.T.);
#51705=EDGE_CURVE('',#37445,#40112,#32908,.T.);
#51706=EDGE_CURVE('',#40099,#37123,#32909,.T.);
#51707=EDGE_CURVE('',#37446,#40111,#32910,.T.);
#51708=EDGE_CURVE('',#40100,#37122,#32911,.T.);
#51709=EDGE_CURVE('',#37447,#40092,#32912,.T.);
#51710=EDGE_CURVE('',#40101,#37814,#32913,.T.);
#51711=EDGE_CURVE('',#37448,#40095,#32914,.T.);
#51712=EDGE_CURVE('',#40102,#37810,#1372,.T.);
#51713=EDGE_CURVE('',#37449,#40098,#32915,.T.);
#51714=EDGE_CURVE('',#40103,#37809,#32916,.T.);
#51715=EDGE_CURVE('',#37450,#40097,#32917,.T.);
#51716=EDGE_CURVE('',#40104,#37806,#32918,.T.);
#51717=EDGE_CURVE('',#37797,#40096,#32919,.T.);
#51718=EDGE_CURVE('',#40105,#37805,#32920,.T.);
#51719=EDGE_CURVE('',#37798,#40107,#1373,.T.);
#51720=EDGE_CURVE('',#40106,#37802,#32921,.T.);
#51721=EDGE_CURVE('',#40147,#37773,#1374,.T.);
#51722=EDGE_CURVE('',#37768,#40146,#32922,.T.);
#51723=EDGE_CURVE('',#37767,#40145,#32923,.T.);
#51724=EDGE_CURVE('',#40136,#37775,#32924,.T.);
#51725=EDGE_CURVE('',#37764,#40144,#32925,.T.);
#51726=EDGE_CURVE('',#40137,#37133,#32926,.T.);
#51727=EDGE_CURVE('',#37763,#40143,#32927,.T.);
#51728=EDGE_CURVE('',#40138,#37132,#32928,.T.);
#51729=EDGE_CURVE('',#37761,#40142,#1375,.T.);
#51730=EDGE_CURVE('',#40121,#37131,#32929,.T.);
#51731=EDGE_CURVE('',#37756,#40141,#32930,.T.);
#51732=EDGE_CURVE('',#40122,#37130,#32931,.T.);
#51733=EDGE_CURVE('',#37439,#40140,#32932,.T.);
#51734=EDGE_CURVE('',#40127,#37129,#32933,.T.);
#51735=EDGE_CURVE('',#37440,#40139,#32934,.T.);
#51736=EDGE_CURVE('',#40128,#37128,#32935,.T.);
#51737=EDGE_CURVE('',#37441,#40120,#32936,.T.);
#51738=EDGE_CURVE('',#40129,#37794,#32937,.T.);
#51739=EDGE_CURVE('',#37442,#40123,#32938,.T.);
#51740=EDGE_CURVE('',#40130,#37790,#1376,.T.);
#51741=EDGE_CURVE('',#37443,#40126,#32939,.T.);
#51742=EDGE_CURVE('',#40131,#37789,#32940,.T.);
#51743=EDGE_CURVE('',#37444,#40125,#32941,.T.);
#51744=EDGE_CURVE('',#40132,#37786,#32942,.T.);
#51745=EDGE_CURVE('',#37777,#40124,#32943,.T.);
#51746=EDGE_CURVE('',#40133,#37785,#32944,.T.);
#51747=EDGE_CURVE('',#37778,#40135,#1377,.T.);
#51748=EDGE_CURVE('',#40134,#37782,#32945,.T.);
#51749=EDGE_CURVE('',#40175,#37753,#1378,.T.);
#51750=EDGE_CURVE('',#37748,#40174,#32946,.T.);
#51751=EDGE_CURVE('',#37747,#40173,#32947,.T.);
#51752=EDGE_CURVE('',#40164,#37755,#32948,.T.);
#51753=EDGE_CURVE('',#37744,#40172,#32949,.T.);
#51754=EDGE_CURVE('',#40165,#37139,#32950,.T.);
#51755=EDGE_CURVE('',#37743,#40171,#32951,.T.);
#51756=EDGE_CURVE('',#40166,#37138,#32952,.T.);
#51757=EDGE_CURVE('',#37741,#40170,#1379,.T.);
#51758=EDGE_CURVE('',#40149,#37137,#32953,.T.);
#51759=EDGE_CURVE('',#37736,#40169,#32954,.T.);
#51760=EDGE_CURVE('',#40150,#37136,#32955,.T.);
#51761=EDGE_CURVE('',#37433,#40168,#32956,.T.);
#51762=EDGE_CURVE('',#40155,#37135,#32957,.T.);
#51763=EDGE_CURVE('',#37434,#40167,#32958,.T.);
#51764=EDGE_CURVE('',#40156,#37134,#32959,.T.);
#51765=EDGE_CURVE('',#37435,#40148,#32960,.T.);
#51766=EDGE_CURVE('',#40157,#37774,#32961,.T.);
#51767=EDGE_CURVE('',#37436,#40151,#32962,.T.);
#51768=EDGE_CURVE('',#40158,#37770,#1380,.T.);
#51769=EDGE_CURVE('',#37437,#40154,#32963,.T.);
#51770=EDGE_CURVE('',#40159,#37769,#32964,.T.);
#51771=EDGE_CURVE('',#37438,#40153,#32965,.T.);
#51772=EDGE_CURVE('',#40160,#37766,#32966,.T.);
#51773=EDGE_CURVE('',#37757,#40152,#32967,.T.);
#51774=EDGE_CURVE('',#40161,#37765,#32968,.T.);
#51775=EDGE_CURVE('',#37758,#40163,#1381,.T.);
#51776=EDGE_CURVE('',#40162,#37762,#32969,.T.);
#51777=EDGE_CURVE('',#40203,#37733,#1382,.T.);
#51778=EDGE_CURVE('',#37728,#40202,#32970,.T.);
#51779=EDGE_CURVE('',#37727,#40201,#32971,.T.);
#51780=EDGE_CURVE('',#40192,#37735,#32972,.T.);
#51781=EDGE_CURVE('',#37724,#40200,#32973,.T.);
#51782=EDGE_CURVE('',#40193,#37145,#32974,.T.);
#51783=EDGE_CURVE('',#37723,#40199,#32975,.T.);
#51784=EDGE_CURVE('',#40194,#37144,#32976,.T.);
#51785=EDGE_CURVE('',#37721,#40198,#1383,.T.);
#51786=EDGE_CURVE('',#40177,#37143,#32977,.T.);
#51787=EDGE_CURVE('',#37716,#40197,#32978,.T.);
#51788=EDGE_CURVE('',#40178,#37142,#32979,.T.);
#51789=EDGE_CURVE('',#37427,#40196,#32980,.T.);
#51790=EDGE_CURVE('',#40183,#37141,#32981,.T.);
#51791=EDGE_CURVE('',#37428,#40195,#32982,.T.);
#51792=EDGE_CURVE('',#40184,#37140,#32983,.T.);
#51793=EDGE_CURVE('',#37429,#40176,#32984,.T.);
#51794=EDGE_CURVE('',#40185,#37754,#32985,.T.);
#51795=EDGE_CURVE('',#37430,#40179,#32986,.T.);
#51796=EDGE_CURVE('',#40186,#37750,#1384,.T.);
#51797=EDGE_CURVE('',#37431,#40182,#32987,.T.);
#51798=EDGE_CURVE('',#40187,#37749,#32988,.T.);
#51799=EDGE_CURVE('',#37432,#40181,#32989,.T.);
#51800=EDGE_CURVE('',#40188,#37746,#32990,.T.);
#51801=EDGE_CURVE('',#37737,#40180,#32991,.T.);
#51802=EDGE_CURVE('',#40189,#37745,#32992,.T.);
#51803=EDGE_CURVE('',#37738,#40191,#1385,.T.);
#51804=EDGE_CURVE('',#40190,#37742,#32993,.T.);
#51805=EDGE_CURVE('',#40231,#37713,#1386,.T.);
#51806=EDGE_CURVE('',#37708,#40230,#32994,.T.);
#51807=EDGE_CURVE('',#37707,#40229,#32995,.T.);
#51808=EDGE_CURVE('',#40220,#37715,#32996,.T.);
#51809=EDGE_CURVE('',#37704,#40228,#32997,.T.);
#51810=EDGE_CURVE('',#40221,#37151,#32998,.T.);
#51811=EDGE_CURVE('',#37703,#40227,#32999,.T.);
#51812=EDGE_CURVE('',#40222,#37150,#33000,.T.);
#51813=EDGE_CURVE('',#37701,#40226,#1387,.T.);
#51814=EDGE_CURVE('',#40205,#37149,#33001,.T.);
#51815=EDGE_CURVE('',#37696,#40225,#33002,.T.);
#51816=EDGE_CURVE('',#40206,#37148,#33003,.T.);
#51817=EDGE_CURVE('',#37421,#40224,#33004,.T.);
#51818=EDGE_CURVE('',#40211,#37147,#33005,.T.);
#51819=EDGE_CURVE('',#37422,#40223,#33006,.T.);
#51820=EDGE_CURVE('',#40212,#37146,#33007,.T.);
#51821=EDGE_CURVE('',#37423,#40204,#33008,.T.);
#51822=EDGE_CURVE('',#40213,#37734,#33009,.T.);
#51823=EDGE_CURVE('',#37424,#40207,#33010,.T.);
#51824=EDGE_CURVE('',#40214,#37730,#1388,.T.);
#51825=EDGE_CURVE('',#37425,#40210,#33011,.T.);
#51826=EDGE_CURVE('',#40215,#37729,#33012,.T.);
#51827=EDGE_CURVE('',#37426,#40209,#33013,.T.);
#51828=EDGE_CURVE('',#40216,#37726,#33014,.T.);
#51829=EDGE_CURVE('',#37717,#40208,#33015,.T.);
#51830=EDGE_CURVE('',#40217,#37725,#33016,.T.);
#51831=EDGE_CURVE('',#37718,#40219,#1389,.T.);
#51832=EDGE_CURVE('',#40218,#37722,#33017,.T.);
#51833=EDGE_CURVE('',#40259,#37693,#1390,.T.);
#51834=EDGE_CURVE('',#37688,#40258,#33018,.T.);
#51835=EDGE_CURVE('',#37687,#40257,#33019,.T.);
#51836=EDGE_CURVE('',#40248,#37695,#33020,.T.);
#51837=EDGE_CURVE('',#37684,#40256,#33021,.T.);
#51838=EDGE_CURVE('',#40249,#37157,#33022,.T.);
#51839=EDGE_CURVE('',#37683,#40255,#33023,.T.);
#51840=EDGE_CURVE('',#40250,#37156,#33024,.T.);
#51841=EDGE_CURVE('',#37681,#40254,#1391,.T.);
#51842=EDGE_CURVE('',#40233,#37155,#33025,.T.);
#51843=EDGE_CURVE('',#37676,#40253,#33026,.T.);
#51844=EDGE_CURVE('',#40234,#37154,#33027,.T.);
#51845=EDGE_CURVE('',#37415,#40252,#33028,.T.);
#51846=EDGE_CURVE('',#40239,#37153,#33029,.T.);
#51847=EDGE_CURVE('',#37416,#40251,#33030,.T.);
#51848=EDGE_CURVE('',#40240,#37152,#33031,.T.);
#51849=EDGE_CURVE('',#37417,#40232,#33032,.T.);
#51850=EDGE_CURVE('',#40241,#37714,#33033,.T.);
#51851=EDGE_CURVE('',#37418,#40235,#33034,.T.);
#51852=EDGE_CURVE('',#40242,#37710,#1392,.T.);
#51853=EDGE_CURVE('',#37419,#40238,#33035,.T.);
#51854=EDGE_CURVE('',#40243,#37709,#33036,.T.);
#51855=EDGE_CURVE('',#37420,#40237,#33037,.T.);
#51856=EDGE_CURVE('',#40244,#37706,#33038,.T.);
#51857=EDGE_CURVE('',#37697,#40236,#33039,.T.);
#51858=EDGE_CURVE('',#40245,#37705,#33040,.T.);
#51859=EDGE_CURVE('',#37698,#40247,#1393,.T.);
#51860=EDGE_CURVE('',#40246,#37702,#33041,.T.);
#51861=EDGE_CURVE('',#40287,#37673,#1394,.T.);
#51862=EDGE_CURVE('',#37668,#40286,#33042,.T.);
#51863=EDGE_CURVE('',#37667,#40285,#33043,.T.);
#51864=EDGE_CURVE('',#40276,#37675,#33044,.T.);
#51865=EDGE_CURVE('',#37664,#40284,#33045,.T.);
#51866=EDGE_CURVE('',#40277,#37163,#33046,.T.);
#51867=EDGE_CURVE('',#37663,#40283,#33047,.T.);
#51868=EDGE_CURVE('',#40278,#37162,#33048,.T.);
#51869=EDGE_CURVE('',#37661,#40282,#1395,.T.);
#51870=EDGE_CURVE('',#40261,#37161,#33049,.T.);
#51871=EDGE_CURVE('',#37656,#40281,#33050,.T.);
#51872=EDGE_CURVE('',#40262,#37160,#33051,.T.);
#51873=EDGE_CURVE('',#37409,#40280,#33052,.T.);
#51874=EDGE_CURVE('',#40267,#37159,#33053,.T.);
#51875=EDGE_CURVE('',#37410,#40279,#33054,.T.);
#51876=EDGE_CURVE('',#40268,#37158,#33055,.T.);
#51877=EDGE_CURVE('',#37411,#40260,#33056,.T.);
#51878=EDGE_CURVE('',#40269,#37694,#33057,.T.);
#51879=EDGE_CURVE('',#37412,#40263,#33058,.T.);
#51880=EDGE_CURVE('',#40270,#37690,#1396,.T.);
#51881=EDGE_CURVE('',#37413,#40266,#33059,.T.);
#51882=EDGE_CURVE('',#40271,#37689,#33060,.T.);
#51883=EDGE_CURVE('',#37414,#40265,#33061,.T.);
#51884=EDGE_CURVE('',#40272,#37686,#33062,.T.);
#51885=EDGE_CURVE('',#37677,#40264,#33063,.T.);
#51886=EDGE_CURVE('',#40273,#37685,#33064,.T.);
#51887=EDGE_CURVE('',#37678,#40275,#1397,.T.);
#51888=EDGE_CURVE('',#40274,#37682,#33065,.T.);
#51889=EDGE_CURVE('',#40315,#37653,#1398,.T.);
#51890=EDGE_CURVE('',#37648,#40314,#33066,.T.);
#51891=EDGE_CURVE('',#37647,#40313,#33067,.T.);
#51892=EDGE_CURVE('',#40304,#37655,#33068,.T.);
#51893=EDGE_CURVE('',#37644,#40312,#33069,.T.);
#51894=EDGE_CURVE('',#40305,#37169,#33070,.T.);
#51895=EDGE_CURVE('',#37643,#40311,#33071,.T.);
#51896=EDGE_CURVE('',#40306,#37168,#33072,.T.);
#51897=EDGE_CURVE('',#37641,#40310,#1399,.T.);
#51898=EDGE_CURVE('',#40289,#37167,#33073,.T.);
#51899=EDGE_CURVE('',#37636,#40309,#33074,.T.);
#51900=EDGE_CURVE('',#40290,#37166,#33075,.T.);
#51901=EDGE_CURVE('',#37403,#40308,#33076,.T.);
#51902=EDGE_CURVE('',#40295,#37165,#33077,.T.);
#51903=EDGE_CURVE('',#37404,#40307,#33078,.T.);
#51904=EDGE_CURVE('',#40296,#37164,#33079,.T.);
#51905=EDGE_CURVE('',#37405,#40288,#33080,.T.);
#51906=EDGE_CURVE('',#40297,#37674,#33081,.T.);
#51907=EDGE_CURVE('',#37406,#40291,#33082,.T.);
#51908=EDGE_CURVE('',#40298,#37670,#1400,.T.);
#51909=EDGE_CURVE('',#37407,#40294,#33083,.T.);
#51910=EDGE_CURVE('',#40299,#37669,#33084,.T.);
#51911=EDGE_CURVE('',#37408,#40293,#33085,.T.);
#51912=EDGE_CURVE('',#40300,#37666,#33086,.T.);
#51913=EDGE_CURVE('',#37657,#40292,#33087,.T.);
#51914=EDGE_CURVE('',#40301,#37665,#33088,.T.);
#51915=EDGE_CURVE('',#37658,#40303,#1401,.T.);
#51916=EDGE_CURVE('',#40302,#37662,#33089,.T.);
#51917=EDGE_CURVE('',#40343,#37633,#1402,.T.);
#51918=EDGE_CURVE('',#37628,#40342,#33090,.T.);
#51919=EDGE_CURVE('',#37627,#40341,#33091,.T.);
#51920=EDGE_CURVE('',#40332,#37635,#33092,.T.);
#51921=EDGE_CURVE('',#37624,#40340,#33093,.T.);
#51922=EDGE_CURVE('',#40333,#37175,#33094,.T.);
#51923=EDGE_CURVE('',#37623,#40339,#33095,.T.);
#51924=EDGE_CURVE('',#40334,#37174,#33096,.T.);
#51925=EDGE_CURVE('',#37621,#40338,#1403,.T.);
#51926=EDGE_CURVE('',#40317,#37173,#33097,.T.);
#51927=EDGE_CURVE('',#37616,#40337,#33098,.T.);
#51928=EDGE_CURVE('',#40318,#37172,#33099,.T.);
#51929=EDGE_CURVE('',#37397,#40336,#33100,.T.);
#51930=EDGE_CURVE('',#40323,#37171,#33101,.T.);
#51931=EDGE_CURVE('',#37398,#40335,#33102,.T.);
#51932=EDGE_CURVE('',#40324,#37170,#33103,.T.);
#51933=EDGE_CURVE('',#37399,#40316,#33104,.T.);
#51934=EDGE_CURVE('',#40325,#37654,#33105,.T.);
#51935=EDGE_CURVE('',#37400,#40319,#33106,.T.);
#51936=EDGE_CURVE('',#40326,#37650,#1404,.T.);
#51937=EDGE_CURVE('',#37401,#40322,#33107,.T.);
#51938=EDGE_CURVE('',#40327,#37649,#33108,.T.);
#51939=EDGE_CURVE('',#37402,#40321,#33109,.T.);
#51940=EDGE_CURVE('',#40328,#37646,#33110,.T.);
#51941=EDGE_CURVE('',#37637,#40320,#33111,.T.);
#51942=EDGE_CURVE('',#40329,#37645,#33112,.T.);
#51943=EDGE_CURVE('',#37638,#40331,#1405,.T.);
#51944=EDGE_CURVE('',#40330,#37642,#33113,.T.);
#51945=EDGE_CURVE('',#40371,#37613,#1406,.T.);
#51946=EDGE_CURVE('',#37608,#40370,#33114,.T.);
#51947=EDGE_CURVE('',#37607,#40369,#33115,.T.);
#51948=EDGE_CURVE('',#40360,#37615,#33116,.T.);
#51949=EDGE_CURVE('',#37604,#40368,#33117,.T.);
#51950=EDGE_CURVE('',#40361,#37181,#33118,.T.);
#51951=EDGE_CURVE('',#37603,#40367,#33119,.T.);
#51952=EDGE_CURVE('',#40362,#37180,#33120,.T.);
#51953=EDGE_CURVE('',#37601,#40366,#1407,.T.);
#51954=EDGE_CURVE('',#40345,#37179,#33121,.T.);
#51955=EDGE_CURVE('',#37596,#40365,#33122,.T.);
#51956=EDGE_CURVE('',#40346,#37178,#33123,.T.);
#51957=EDGE_CURVE('',#37391,#40364,#33124,.T.);
#51958=EDGE_CURVE('',#40351,#37177,#33125,.T.);
#51959=EDGE_CURVE('',#37392,#40363,#33126,.T.);
#51960=EDGE_CURVE('',#40352,#37176,#33127,.T.);
#51961=EDGE_CURVE('',#37393,#40344,#33128,.T.);
#51962=EDGE_CURVE('',#40353,#37634,#33129,.T.);
#51963=EDGE_CURVE('',#37394,#40347,#33130,.T.);
#51964=EDGE_CURVE('',#40354,#37630,#1408,.T.);
#51965=EDGE_CURVE('',#37395,#40350,#33131,.T.);
#51966=EDGE_CURVE('',#40355,#37629,#33132,.T.);
#51967=EDGE_CURVE('',#37396,#40349,#33133,.T.);
#51968=EDGE_CURVE('',#40356,#37626,#33134,.T.);
#51969=EDGE_CURVE('',#37617,#40348,#33135,.T.);
#51970=EDGE_CURVE('',#40357,#37625,#33136,.T.);
#51971=EDGE_CURVE('',#37618,#40359,#1409,.T.);
#51972=EDGE_CURVE('',#40358,#37622,#33137,.T.);
#51973=EDGE_CURVE('',#40399,#37593,#1410,.T.);
#51974=EDGE_CURVE('',#37588,#40398,#33138,.T.);
#51975=EDGE_CURVE('',#37587,#40397,#33139,.T.);
#51976=EDGE_CURVE('',#40388,#37595,#33140,.T.);
#51977=EDGE_CURVE('',#37584,#40396,#33141,.T.);
#51978=EDGE_CURVE('',#40389,#37187,#33142,.T.);
#51979=EDGE_CURVE('',#37583,#40395,#33143,.T.);
#51980=EDGE_CURVE('',#40390,#37186,#33144,.T.);
#51981=EDGE_CURVE('',#37581,#40394,#1411,.T.);
#51982=EDGE_CURVE('',#40373,#37185,#33145,.T.);
#51983=EDGE_CURVE('',#37576,#40393,#33146,.T.);
#51984=EDGE_CURVE('',#40374,#37184,#33147,.T.);
#51985=EDGE_CURVE('',#37385,#40392,#33148,.T.);
#51986=EDGE_CURVE('',#40379,#37183,#33149,.T.);
#51987=EDGE_CURVE('',#37386,#40391,#33150,.T.);
#51988=EDGE_CURVE('',#40380,#37182,#33151,.T.);
#51989=EDGE_CURVE('',#37387,#40372,#33152,.T.);
#51990=EDGE_CURVE('',#40381,#37614,#33153,.T.);
#51991=EDGE_CURVE('',#37388,#40375,#33154,.T.);
#51992=EDGE_CURVE('',#40382,#37610,#1412,.T.);
#51993=EDGE_CURVE('',#37389,#40378,#33155,.T.);
#51994=EDGE_CURVE('',#40383,#37609,#33156,.T.);
#51995=EDGE_CURVE('',#37390,#40377,#33157,.T.);
#51996=EDGE_CURVE('',#40384,#37606,#33158,.T.);
#51997=EDGE_CURVE('',#37597,#40376,#33159,.T.);
#51998=EDGE_CURVE('',#40385,#37605,#33160,.T.);
#51999=EDGE_CURVE('',#37598,#40387,#1413,.T.);
#52000=EDGE_CURVE('',#40386,#37602,#33161,.T.);
#52001=EDGE_CURVE('',#40427,#37568,#1414,.T.);
#52002=EDGE_CURVE('',#37570,#40426,#33162,.T.);
#52003=EDGE_CURVE('',#37565,#40425,#33163,.T.);
#52004=EDGE_CURVE('',#40416,#37575,#33164,.T.);
#52005=EDGE_CURVE('',#37566,#40424,#33165,.T.);
#52006=EDGE_CURVE('',#40417,#37193,#33166,.T.);
#52007=EDGE_CURVE('',#37563,#40423,#33167,.T.);
#52008=EDGE_CURVE('',#40418,#37192,#33168,.T.);
#52009=EDGE_CURVE('',#37556,#40422,#1415,.T.);
#52010=EDGE_CURVE('',#40401,#37191,#33169,.T.);
#52011=EDGE_CURVE('',#37558,#40421,#33170,.T.);
#52012=EDGE_CURVE('',#40402,#37190,#33171,.T.);
#52013=EDGE_CURVE('',#37379,#40420,#33172,.T.);
#52014=EDGE_CURVE('',#40407,#37189,#33173,.T.);
#52015=EDGE_CURVE('',#37380,#40419,#33174,.T.);
#52016=EDGE_CURVE('',#40408,#37188,#33175,.T.);
#52017=EDGE_CURVE('',#37381,#40400,#33176,.T.);
#52018=EDGE_CURVE('',#40409,#37594,#33177,.T.);
#52019=EDGE_CURVE('',#37382,#40403,#33178,.T.);
#52020=EDGE_CURVE('',#40410,#37590,#1416,.T.);
#52021=EDGE_CURVE('',#37383,#40406,#33179,.T.);
#52022=EDGE_CURVE('',#40411,#37589,#33180,.T.);
#52023=EDGE_CURVE('',#37384,#40405,#33181,.T.);
#52024=EDGE_CURVE('',#40412,#37586,#33182,.T.);
#52025=EDGE_CURVE('',#37577,#40404,#33183,.T.);
#52026=EDGE_CURVE('',#40413,#37585,#33184,.T.);
#52027=EDGE_CURVE('',#37578,#40415,#1417,.T.);
#52028=EDGE_CURVE('',#40414,#37582,#33185,.T.);
#52029=EDGE_CURVE('',#40428,#40429,#33186,.T.);
#52030=EDGE_CURVE('',#40430,#40428,#33187,.T.);
#52031=EDGE_CURVE('',#40431,#40430,#33188,.T.);
#52032=EDGE_CURVE('',#40431,#40429,#33189,.T.);
#52033=EDGE_CURVE('',#40432,#40433,#33190,.T.);
#52034=EDGE_CURVE('',#40434,#40432,#33191,.T.);
#52035=EDGE_CURVE('',#40435,#40434,#33192,.T.);
#52036=EDGE_CURVE('',#40435,#40433,#33193,.T.);
#52037=EDGE_CURVE('',#40436,#40437,#33194,.T.);
#52038=EDGE_CURVE('',#40438,#40436,#33195,.T.);
#52039=EDGE_CURVE('',#40439,#40438,#33196,.T.);
#52040=EDGE_CURVE('',#40439,#40437,#33197,.T.);
#52041=EDGE_CURVE('',#40440,#40441,#33198,.T.);
#52042=EDGE_CURVE('',#40442,#40440,#33199,.T.);
#52043=EDGE_CURVE('',#40443,#40442,#33200,.T.);
#52044=EDGE_CURVE('',#40443,#40444,#33201,.T.);
#52045=EDGE_CURVE('',#40441,#40444,#33202,.T.);
#52046=EDGE_CURVE('',#40445,#40445,#33203,.T.);
#52047=EDGE_CURVE('',#40445,#40446,#33204,.T.);
#52048=EDGE_CURVE('',#40447,#40446,#33205,.T.);
#52049=EDGE_CURVE('',#40446,#40447,#33206,.T.);
#52050=EDGE_CURVE('',#40448,#40448,#33207,.T.);
#52051=EDGE_CURVE('',#40448,#40449,#33208,.T.);
#52052=EDGE_CURVE('',#40449,#40449,#33209,.T.);
#52053=EDGE_CURVE('',#40450,#40450,#33210,.T.);
#52054=EDGE_CURVE('',#40450,#40451,#33211,.T.);
#52055=EDGE_CURVE('',#40452,#40451,#33212,.T.);
#52056=EDGE_CURVE('',#40451,#40452,#33213,.T.);
#52057=EDGE_CURVE('',#40453,#40453,#33214,.T.);
#52058=EDGE_CURVE('',#40453,#40454,#33215,.T.);
#52059=EDGE_CURVE('',#40454,#40454,#33216,.T.);
#52060=EDGE_CURVE('',#40455,#40455,#33217,.T.);
#52061=EDGE_CURVE('',#40455,#40456,#22034,.T.);
#52062=EDGE_CURVE('',#40456,#40456,#33218,.T.);
#52063=EDGE_CURVE('',#40456,#40453,#22035,.T.);
#52064=EDGE_CURVE('',#40457,#40458,#33219,.T.);
#52065=EDGE_CURVE('',#40458,#40459,#4735,.T.);
#52066=EDGE_CURVE('',#40459,#40460,#22036,.T.);
#52067=EDGE_CURVE('',#40460,#40461,#33220,.T.);
#52068=EDGE_CURVE('',#40461,#40462,#22037,.T.);
#52069=EDGE_CURVE('',#40462,#40463,#4736,.T.);
#52070=EDGE_CURVE('',#40463,#40464,#33221,.T.);
#52071=EDGE_CURVE('',#40464,#40465,#4737,.T.);
#52072=EDGE_CURVE('',#40465,#40466,#22038,.T.);
#52073=EDGE_CURVE('',#40466,#40467,#33222,.T.);
#52074=EDGE_CURVE('',#40467,#40468,#22039,.T.);
#52075=EDGE_CURVE('',#40468,#40469,#4738,.T.);
#52076=EDGE_CURVE('',#40469,#40470,#33223,.T.);
#52077=EDGE_CURVE('',#40470,#40471,#4739,.T.);
#52078=EDGE_CURVE('',#40471,#40472,#22040,.T.);
#52079=EDGE_CURVE('',#40472,#40473,#33224,.T.);
#52080=EDGE_CURVE('',#40473,#40474,#22041,.T.);
#52081=EDGE_CURVE('',#40474,#40475,#4740,.T.);
#52082=EDGE_CURVE('',#40475,#40476,#33225,.T.);
#52083=EDGE_CURVE('',#40476,#40477,#4741,.T.);
#52084=EDGE_CURVE('',#40477,#40478,#22042,.T.);
#52085=EDGE_CURVE('',#40478,#40479,#33226,.T.);
#52086=EDGE_CURVE('',#40479,#40480,#22043,.T.);
#52087=EDGE_CURVE('',#40480,#40481,#4742,.T.);
#52088=EDGE_CURVE('',#40481,#40482,#33227,.T.);
#52089=EDGE_CURVE('',#40482,#40483,#4743,.T.);
#52090=EDGE_CURVE('',#40483,#40484,#22044,.T.);
#52091=EDGE_CURVE('',#40484,#40485,#33228,.T.);
#52092=EDGE_CURVE('',#40485,#40486,#22045,.T.);
#52093=EDGE_CURVE('',#40486,#40487,#4744,.T.);
#52094=EDGE_CURVE('',#40487,#40488,#33229,.T.);
#52095=EDGE_CURVE('',#40488,#40489,#4745,.T.);
#52096=EDGE_CURVE('',#40489,#40490,#22046,.T.);
#52097=EDGE_CURVE('',#40490,#40491,#33230,.T.);
#52098=EDGE_CURVE('',#40491,#40492,#22047,.T.);
#52099=EDGE_CURVE('',#40492,#40493,#4746,.T.);
#52100=EDGE_CURVE('',#40493,#40494,#33231,.T.);
#52101=EDGE_CURVE('',#40494,#40495,#4747,.T.);
#52102=EDGE_CURVE('',#40495,#40496,#22048,.T.);
#52103=EDGE_CURVE('',#40496,#40497,#33232,.T.);
#52104=EDGE_CURVE('',#40497,#40498,#22049,.T.);
#52105=EDGE_CURVE('',#40498,#40499,#4748,.T.);
#52106=EDGE_CURVE('',#40499,#40500,#33233,.T.);
#52107=EDGE_CURVE('',#40500,#40501,#4749,.T.);
#52108=EDGE_CURVE('',#40501,#40502,#22050,.T.);
#52109=EDGE_CURVE('',#40502,#40503,#33234,.T.);
#52110=EDGE_CURVE('',#40503,#40504,#22051,.T.);
#52111=EDGE_CURVE('',#40504,#40505,#4750,.T.);
#52112=EDGE_CURVE('',#40505,#40506,#33235,.T.);
#52113=EDGE_CURVE('',#40506,#40507,#4751,.T.);
#52114=EDGE_CURVE('',#40507,#40508,#22052,.T.);
#52115=EDGE_CURVE('',#40508,#40509,#33236,.T.);
#52116=EDGE_CURVE('',#40509,#40510,#22053,.T.);
#52117=EDGE_CURVE('',#40510,#40511,#4752,.T.);
#52118=EDGE_CURVE('',#40511,#40512,#33237,.T.);
#52119=EDGE_CURVE('',#40512,#40513,#4753,.T.);
#52120=EDGE_CURVE('',#40513,#40514,#22054,.T.);
#52121=EDGE_CURVE('',#40514,#40515,#33238,.T.);
#52122=EDGE_CURVE('',#40515,#40516,#22055,.T.);
#52123=EDGE_CURVE('',#40516,#40517,#4754,.T.);
#52124=EDGE_CURVE('',#40517,#40518,#33239,.T.);
#52125=EDGE_CURVE('',#40518,#40519,#4755,.T.);
#52126=EDGE_CURVE('',#40519,#40520,#22056,.T.);
#52127=EDGE_CURVE('',#40520,#40521,#33240,.T.);
#52128=EDGE_CURVE('',#40521,#40522,#22057,.T.);
#52129=EDGE_CURVE('',#40522,#40523,#4756,.T.);
#52130=EDGE_CURVE('',#40523,#40524,#33241,.T.);
#52131=EDGE_CURVE('',#40524,#40525,#4757,.T.);
#52132=EDGE_CURVE('',#40525,#40526,#22058,.T.);
#52133=EDGE_CURVE('',#40526,#40527,#33242,.T.);
#52134=EDGE_CURVE('',#40527,#40528,#22059,.T.);
#52135=EDGE_CURVE('',#40528,#40529,#4758,.T.);
#52136=EDGE_CURVE('',#40529,#40530,#33243,.T.);
#52137=EDGE_CURVE('',#40530,#40531,#4759,.T.);
#52138=EDGE_CURVE('',#40531,#40532,#22060,.T.);
#52139=EDGE_CURVE('',#40532,#40533,#33244,.T.);
#52140=EDGE_CURVE('',#40533,#40534,#22061,.T.);
#52141=EDGE_CURVE('',#40534,#40535,#4760,.T.);
#52142=EDGE_CURVE('',#40535,#40536,#33245,.T.);
#52143=EDGE_CURVE('',#40536,#40537,#4761,.T.);
#52144=EDGE_CURVE('',#40537,#40538,#22062,.T.);
#52145=EDGE_CURVE('',#40538,#40539,#33246,.T.);
#52146=EDGE_CURVE('',#40539,#40540,#22063,.T.);
#52147=EDGE_CURVE('',#40540,#40541,#4762,.T.);
#52148=EDGE_CURVE('',#40541,#40542,#33247,.T.);
#52149=EDGE_CURVE('',#40542,#40543,#4763,.T.);
#52150=EDGE_CURVE('',#40543,#40544,#22064,.T.);
#52151=EDGE_CURVE('',#40544,#40545,#33248,.T.);
#52152=EDGE_CURVE('',#40545,#40546,#22065,.T.);
#52153=EDGE_CURVE('',#40546,#40547,#4764,.T.);
#52154=EDGE_CURVE('',#40547,#40548,#33249,.T.);
#52155=EDGE_CURVE('',#40548,#40549,#4765,.T.);
#52156=EDGE_CURVE('',#40549,#40550,#22066,.T.);
#52157=EDGE_CURVE('',#40550,#40551,#33250,.T.);
#52158=EDGE_CURVE('',#40551,#40552,#22067,.T.);
#52159=EDGE_CURVE('',#40552,#40553,#4766,.T.);
#52160=EDGE_CURVE('',#40553,#40554,#33251,.T.);
#52161=EDGE_CURVE('',#40554,#40555,#4767,.T.);
#52162=EDGE_CURVE('',#40555,#40556,#22068,.T.);
#52163=EDGE_CURVE('',#40556,#40557,#33252,.T.);
#52164=EDGE_CURVE('',#40557,#40558,#22069,.T.);
#52165=EDGE_CURVE('',#40558,#40559,#4768,.T.);
#52166=EDGE_CURVE('',#40559,#40560,#33253,.T.);
#52167=EDGE_CURVE('',#40560,#40561,#4769,.T.);
#52168=EDGE_CURVE('',#40561,#40562,#22070,.T.);
#52169=EDGE_CURVE('',#40562,#40563,#33254,.T.);
#52170=EDGE_CURVE('',#40563,#40564,#22071,.T.);
#52171=EDGE_CURVE('',#40564,#40565,#4770,.T.);
#52172=EDGE_CURVE('',#40565,#40566,#33255,.T.);
#52173=EDGE_CURVE('',#40566,#40567,#4771,.T.);
#52174=EDGE_CURVE('',#40567,#40568,#22072,.T.);
#52175=EDGE_CURVE('',#40568,#40569,#33256,.T.);
#52176=EDGE_CURVE('',#40569,#40570,#22073,.T.);
#52177=EDGE_CURVE('',#40570,#40571,#4772,.T.);
#52178=EDGE_CURVE('',#40571,#40572,#33257,.T.);
#52179=EDGE_CURVE('',#40572,#40573,#4773,.T.);
#52180=EDGE_CURVE('',#40573,#40574,#22074,.T.);
#52181=EDGE_CURVE('',#40574,#40575,#33258,.T.);
#52182=EDGE_CURVE('',#40575,#40576,#22075,.T.);
#52183=EDGE_CURVE('',#40576,#40577,#4774,.T.);
#52184=EDGE_CURVE('',#40577,#40578,#33259,.T.);
#52185=EDGE_CURVE('',#40578,#40579,#4775,.T.);
#52186=EDGE_CURVE('',#40579,#40580,#22076,.T.);
#52187=EDGE_CURVE('',#40580,#40581,#33260,.T.);
#52188=EDGE_CURVE('',#40581,#40582,#22077,.T.);
#52189=EDGE_CURVE('',#40582,#40583,#4776,.T.);
#52190=EDGE_CURVE('',#40583,#40584,#33261,.T.);
#52191=EDGE_CURVE('',#40584,#40585,#4777,.T.);
#52192=EDGE_CURVE('',#40585,#40586,#22078,.T.);
#52193=EDGE_CURVE('',#40586,#40587,#33262,.T.);
#52194=EDGE_CURVE('',#40587,#40588,#22079,.T.);
#52195=EDGE_CURVE('',#40588,#40589,#4778,.T.);
#52196=EDGE_CURVE('',#40589,#40590,#33263,.T.);
#52197=EDGE_CURVE('',#40590,#40591,#4779,.T.);
#52198=EDGE_CURVE('',#40591,#40592,#22080,.T.);
#52199=EDGE_CURVE('',#40592,#40593,#33264,.T.);
#52200=EDGE_CURVE('',#40593,#40594,#22081,.T.);
#52201=EDGE_CURVE('',#40594,#40595,#4780,.T.);
#52202=EDGE_CURVE('',#40595,#40596,#33265,.T.);
#52203=EDGE_CURVE('',#40596,#40597,#4781,.T.);
#52204=EDGE_CURVE('',#40597,#40598,#22082,.T.);
#52205=EDGE_CURVE('',#40598,#40599,#33266,.T.);
#52206=EDGE_CURVE('',#40599,#40600,#22083,.T.);
#52207=EDGE_CURVE('',#40600,#40601,#4782,.T.);
#52208=EDGE_CURVE('',#40601,#40602,#33267,.T.);
#52209=EDGE_CURVE('',#40602,#40603,#4783,.T.);
#52210=EDGE_CURVE('',#40603,#40604,#22084,.T.);
#52211=EDGE_CURVE('',#40604,#40605,#33268,.T.);
#52212=EDGE_CURVE('',#40605,#40606,#22085,.T.);
#52213=EDGE_CURVE('',#40606,#40607,#4784,.T.);
#52214=EDGE_CURVE('',#40607,#40608,#33269,.T.);
#52215=EDGE_CURVE('',#40608,#40609,#4785,.T.);
#52216=EDGE_CURVE('',#40609,#40610,#22086,.T.);
#52217=EDGE_CURVE('',#40610,#40611,#33270,.T.);
#52218=EDGE_CURVE('',#40611,#40612,#22087,.T.);
#52219=EDGE_CURVE('',#40612,#40613,#4786,.T.);
#52220=EDGE_CURVE('',#40613,#40614,#33271,.T.);
#52221=EDGE_CURVE('',#40614,#40615,#4787,.T.);
#52222=EDGE_CURVE('',#40615,#40616,#22088,.T.);
#52223=EDGE_CURVE('',#40616,#40617,#33272,.T.);
#52224=EDGE_CURVE('',#40617,#40618,#22089,.T.);
#52225=EDGE_CURVE('',#40618,#40619,#4788,.T.);
#52226=EDGE_CURVE('',#40619,#40620,#33273,.T.);
#52227=EDGE_CURVE('',#40620,#40621,#4789,.T.);
#52228=EDGE_CURVE('',#40621,#40622,#22090,.T.);
#52229=EDGE_CURVE('',#40622,#40623,#33274,.T.);
#52230=EDGE_CURVE('',#40623,#40624,#22091,.T.);
#52231=EDGE_CURVE('',#40624,#40625,#4790,.T.);
#52232=EDGE_CURVE('',#40625,#40626,#33275,.T.);
#52233=EDGE_CURVE('',#40626,#40627,#4791,.T.);
#52234=EDGE_CURVE('',#40627,#40628,#22092,.T.);
#52235=EDGE_CURVE('',#40628,#40629,#33276,.T.);
#52236=EDGE_CURVE('',#40629,#40630,#22093,.T.);
#52237=EDGE_CURVE('',#40630,#40631,#4792,.T.);
#52238=EDGE_CURVE('',#40631,#40632,#33277,.T.);
#52239=EDGE_CURVE('',#40632,#40633,#4793,.T.);
#52240=EDGE_CURVE('',#40633,#40634,#22094,.T.);
#52241=EDGE_CURVE('',#40634,#40635,#33278,.T.);
#52242=EDGE_CURVE('',#40635,#40636,#22095,.T.);
#52243=EDGE_CURVE('',#40636,#40440,#4794,.T.);
#52244=EDGE_CURVE('',#40441,#40452,#22096,.T.);
#52245=EDGE_CURVE('',#40444,#40637,#4795,.T.);
#52246=EDGE_CURVE('',#40637,#40638,#22097,.T.);
#52247=EDGE_CURVE('',#40638,#40639,#33279,.T.);
#52248=EDGE_CURVE('',#40639,#40640,#22098,.T.);
#52249=EDGE_CURVE('',#40640,#40641,#4796,.T.);
#52250=EDGE_CURVE('',#40641,#40642,#33280,.T.);
#52251=EDGE_CURVE('',#40642,#40643,#4797,.T.);
#52252=EDGE_CURVE('',#40643,#40644,#22099,.T.);
#52253=EDGE_CURVE('',#40644,#40645,#33281,.T.);
#52254=EDGE_CURVE('',#40645,#40646,#22100,.T.);
#52255=EDGE_CURVE('',#40646,#40647,#4798,.T.);
#52256=EDGE_CURVE('',#40647,#40648,#33282,.T.);
#52257=EDGE_CURVE('',#40648,#40649,#4799,.T.);
#52258=EDGE_CURVE('',#40649,#40650,#22101,.T.);
#52259=EDGE_CURVE('',#40650,#40651,#33283,.T.);
#52260=EDGE_CURVE('',#40651,#40652,#22102,.T.);
#52261=EDGE_CURVE('',#40652,#40653,#4800,.T.);
#52262=EDGE_CURVE('',#40653,#40654,#33284,.T.);
#52263=EDGE_CURVE('',#40654,#40655,#4801,.T.);
#52264=EDGE_CURVE('',#40655,#40656,#22103,.T.);
#52265=EDGE_CURVE('',#40656,#40657,#33285,.T.);
#52266=EDGE_CURVE('',#40657,#40658,#22104,.T.);
#52267=EDGE_CURVE('',#40658,#40659,#4802,.T.);
#52268=EDGE_CURVE('',#40659,#40660,#33286,.T.);
#52269=EDGE_CURVE('',#40660,#40661,#4803,.T.);
#52270=EDGE_CURVE('',#40661,#40662,#22105,.T.);
#52271=EDGE_CURVE('',#40662,#40663,#33287,.T.);
#52272=EDGE_CURVE('',#40663,#40664,#22106,.T.);
#52273=EDGE_CURVE('',#40664,#40665,#4804,.T.);
#52274=EDGE_CURVE('',#40665,#40666,#33288,.T.);
#52275=EDGE_CURVE('',#40666,#40667,#4805,.T.);
#52276=EDGE_CURVE('',#40667,#40668,#22107,.T.);
#52277=EDGE_CURVE('',#40668,#40669,#33289,.T.);
#52278=EDGE_CURVE('',#40669,#40670,#22108,.T.);
#52279=EDGE_CURVE('',#40670,#40671,#4806,.T.);
#52280=EDGE_CURVE('',#40671,#40672,#33290,.T.);
#52281=EDGE_CURVE('',#40672,#40673,#4807,.T.);
#52282=EDGE_CURVE('',#40673,#40674,#22109,.T.);
#52283=EDGE_CURVE('',#40674,#40675,#33291,.T.);
#52284=EDGE_CURVE('',#40675,#40676,#22110,.T.);
#52285=EDGE_CURVE('',#40676,#40677,#4808,.T.);
#52286=EDGE_CURVE('',#40677,#40678,#33292,.T.);
#52287=EDGE_CURVE('',#40678,#40679,#4809,.T.);
#52288=EDGE_CURVE('',#40679,#40680,#22111,.T.);
#52289=EDGE_CURVE('',#40680,#40681,#33293,.T.);
#52290=EDGE_CURVE('',#40681,#40682,#22112,.T.);
#52291=EDGE_CURVE('',#40682,#40683,#4810,.T.);
#52292=EDGE_CURVE('',#40683,#40684,#33294,.T.);
#52293=EDGE_CURVE('',#40684,#40685,#4811,.T.);
#52294=EDGE_CURVE('',#40685,#40686,#22113,.T.);
#52295=EDGE_CURVE('',#40686,#40687,#33295,.T.);
#52296=EDGE_CURVE('',#40687,#40688,#22114,.T.);
#52297=EDGE_CURVE('',#40688,#40689,#4812,.T.);
#52298=EDGE_CURVE('',#40689,#40690,#33296,.T.);
#52299=EDGE_CURVE('',#40690,#40691,#4813,.T.);
#52300=EDGE_CURVE('',#40691,#40692,#22115,.T.);
#52301=EDGE_CURVE('',#40692,#40693,#33297,.T.);
#52302=EDGE_CURVE('',#40693,#40694,#22116,.T.);
#52303=EDGE_CURVE('',#40694,#40695,#4814,.T.);
#52304=EDGE_CURVE('',#40695,#40696,#33298,.T.);
#52305=EDGE_CURVE('',#40696,#40697,#4815,.T.);
#52306=EDGE_CURVE('',#40697,#40698,#22117,.T.);
#52307=EDGE_CURVE('',#40698,#40699,#33299,.T.);
#52308=EDGE_CURVE('',#40699,#40700,#22118,.T.);
#52309=EDGE_CURVE('',#40700,#40701,#4816,.T.);
#52310=EDGE_CURVE('',#40701,#40702,#33300,.T.);
#52311=EDGE_CURVE('',#40702,#40703,#4817,.T.);
#52312=EDGE_CURVE('',#40703,#40704,#22119,.T.);
#52313=EDGE_CURVE('',#40704,#40705,#33301,.T.);
#52314=EDGE_CURVE('',#40705,#40706,#22120,.T.);
#52315=EDGE_CURVE('',#40706,#40707,#4818,.T.);
#52316=EDGE_CURVE('',#40707,#40708,#33302,.T.);
#52317=EDGE_CURVE('',#40708,#40709,#4819,.T.);
#52318=EDGE_CURVE('',#40709,#40710,#22121,.T.);
#52319=EDGE_CURVE('',#40710,#40711,#33303,.T.);
#52320=EDGE_CURVE('',#40711,#40712,#22122,.T.);
#52321=EDGE_CURVE('',#40712,#40713,#4820,.T.);
#52322=EDGE_CURVE('',#40713,#40714,#33304,.T.);
#52323=EDGE_CURVE('',#40714,#40715,#4821,.T.);
#52324=EDGE_CURVE('',#40715,#40716,#22123,.T.);
#52325=EDGE_CURVE('',#40716,#40717,#33305,.T.);
#52326=EDGE_CURVE('',#40717,#40718,#22124,.T.);
#52327=EDGE_CURVE('',#40718,#40719,#4822,.T.);
#52328=EDGE_CURVE('',#40719,#40720,#33306,.T.);
#52329=EDGE_CURVE('',#40720,#40721,#4823,.T.);
#52330=EDGE_CURVE('',#40721,#40722,#22125,.T.);
#52331=EDGE_CURVE('',#40722,#40723,#33307,.T.);
#52332=EDGE_CURVE('',#40723,#40724,#22126,.T.);
#52333=EDGE_CURVE('',#40724,#40432,#4824,.T.);
#52334=EDGE_CURVE('',#40433,#40725,#4825,.T.);
#52335=EDGE_CURVE('',#40725,#40726,#22127,.T.);
#52336=EDGE_CURVE('',#40726,#40727,#33308,.T.);
#52337=EDGE_CURVE('',#40727,#40728,#22128,.T.);
#52338=EDGE_CURVE('',#40728,#40729,#4826,.T.);
#52339=EDGE_CURVE('',#40729,#40730,#33309,.T.);
#52340=EDGE_CURVE('',#40730,#40731,#4827,.T.);
#52341=EDGE_CURVE('',#40731,#40732,#22129,.T.);
#52342=EDGE_CURVE('',#40732,#40733,#33310,.T.);
#52343=EDGE_CURVE('',#40733,#40734,#22130,.T.);
#52344=EDGE_CURVE('',#40734,#40735,#4828,.T.);
#52345=EDGE_CURVE('',#40735,#40736,#33311,.T.);
#52346=EDGE_CURVE('',#40736,#40737,#4829,.T.);
#52347=EDGE_CURVE('',#40737,#40738,#22131,.T.);
#52348=EDGE_CURVE('',#40738,#40739,#33312,.T.);
#52349=EDGE_CURVE('',#40739,#40740,#22132,.T.);
#52350=EDGE_CURVE('',#40740,#40741,#4830,.T.);
#52351=EDGE_CURVE('',#40741,#40742,#33313,.T.);
#52352=EDGE_CURVE('',#40742,#40743,#4831,.T.);
#52353=EDGE_CURVE('',#40743,#40744,#22133,.T.);
#52354=EDGE_CURVE('',#40744,#40745,#33314,.T.);
#52355=EDGE_CURVE('',#40745,#40746,#22134,.T.);
#52356=EDGE_CURVE('',#40746,#40747,#4832,.T.);
#52357=EDGE_CURVE('',#40747,#40748,#33315,.T.);
#52358=EDGE_CURVE('',#40748,#40749,#4833,.T.);
#52359=EDGE_CURVE('',#40749,#40750,#22135,.T.);
#52360=EDGE_CURVE('',#40750,#40751,#33316,.T.);
#52361=EDGE_CURVE('',#40751,#40752,#22136,.T.);
#52362=EDGE_CURVE('',#40752,#40753,#4834,.T.);
#52363=EDGE_CURVE('',#40753,#40754,#33317,.T.);
#52364=EDGE_CURVE('',#40754,#40755,#4835,.T.);
#52365=EDGE_CURVE('',#40755,#40756,#22137,.T.);
#52366=EDGE_CURVE('',#40756,#40757,#33318,.T.);
#52367=EDGE_CURVE('',#40757,#40758,#22138,.T.);
#52368=EDGE_CURVE('',#40758,#40759,#4836,.T.);
#52369=EDGE_CURVE('',#40759,#40760,#33319,.T.);
#52370=EDGE_CURVE('',#40760,#40761,#4837,.T.);
#52371=EDGE_CURVE('',#40761,#40762,#22139,.T.);
#52372=EDGE_CURVE('',#40762,#40763,#33320,.T.);
#52373=EDGE_CURVE('',#40763,#40764,#22140,.T.);
#52374=EDGE_CURVE('',#40764,#40765,#4838,.T.);
#52375=EDGE_CURVE('',#40765,#40766,#33321,.T.);
#52376=EDGE_CURVE('',#40766,#40767,#4839,.T.);
#52377=EDGE_CURVE('',#40767,#40768,#22141,.T.);
#52378=EDGE_CURVE('',#40768,#40769,#33322,.T.);
#52379=EDGE_CURVE('',#40769,#40770,#22142,.T.);
#52380=EDGE_CURVE('',#40770,#40771,#4840,.T.);
#52381=EDGE_CURVE('',#40771,#40772,#33323,.T.);
#52382=EDGE_CURVE('',#40772,#40773,#4841,.T.);
#52383=EDGE_CURVE('',#40773,#40774,#22143,.T.);
#52384=EDGE_CURVE('',#40774,#40775,#33324,.T.);
#52385=EDGE_CURVE('',#40775,#40776,#22144,.T.);
#52386=EDGE_CURVE('',#40776,#40777,#4842,.T.);
#52387=EDGE_CURVE('',#40777,#40778,#33325,.T.);
#52388=EDGE_CURVE('',#40778,#40779,#4843,.T.);
#52389=EDGE_CURVE('',#40779,#40780,#22145,.T.);
#52390=EDGE_CURVE('',#40780,#40781,#33326,.T.);
#52391=EDGE_CURVE('',#40781,#40782,#22146,.T.);
#52392=EDGE_CURVE('',#40782,#40783,#4844,.T.);
#52393=EDGE_CURVE('',#40783,#40784,#33327,.T.);
#52394=EDGE_CURVE('',#40784,#40785,#4845,.T.);
#52395=EDGE_CURVE('',#40785,#40786,#22147,.T.);
#52396=EDGE_CURVE('',#40786,#40787,#33328,.T.);
#52397=EDGE_CURVE('',#40787,#40788,#22148,.T.);
#52398=EDGE_CURVE('',#40788,#40789,#4846,.T.);
#52399=EDGE_CURVE('',#40789,#40790,#33329,.T.);
#52400=EDGE_CURVE('',#40790,#40791,#4847,.T.);
#52401=EDGE_CURVE('',#40791,#40792,#22149,.T.);
#52402=EDGE_CURVE('',#40792,#40793,#33330,.T.);
#52403=EDGE_CURVE('',#40793,#40794,#22150,.T.);
#52404=EDGE_CURVE('',#40794,#40795,#4848,.T.);
#52405=EDGE_CURVE('',#40795,#40796,#33331,.T.);
#52406=EDGE_CURVE('',#40796,#40797,#4849,.T.);
#52407=EDGE_CURVE('',#40797,#40798,#22151,.T.);
#52408=EDGE_CURVE('',#40798,#40799,#33332,.T.);
#52409=EDGE_CURVE('',#40799,#40800,#22152,.T.);
#52410=EDGE_CURVE('',#40800,#40801,#4850,.T.);
#52411=EDGE_CURVE('',#40801,#40802,#33333,.T.);
#52412=EDGE_CURVE('',#40802,#40803,#4851,.T.);
#52413=EDGE_CURVE('',#40803,#40804,#22153,.T.);
#52414=EDGE_CURVE('',#40804,#40805,#33334,.T.);
#52415=EDGE_CURVE('',#40805,#40806,#22154,.T.);
#52416=EDGE_CURVE('',#40806,#40807,#4852,.T.);
#52417=EDGE_CURVE('',#40807,#40808,#33335,.T.);
#52418=EDGE_CURVE('',#40808,#40809,#4853,.T.);
#52419=EDGE_CURVE('',#40809,#40810,#22155,.T.);
#52420=EDGE_CURVE('',#40810,#40811,#33336,.T.);
#52421=EDGE_CURVE('',#40811,#40812,#22156,.T.);
#52422=EDGE_CURVE('',#40812,#40457,#4854,.T.);
#52423=EDGE_CURVE('',#40438,#40813,#4855,.T.);
#52424=EDGE_CURVE('',#40813,#40814,#22157,.T.);
#52425=EDGE_CURVE('',#40814,#40815,#33337,.T.);
#52426=EDGE_CURVE('',#40815,#40816,#22158,.T.);
#52427=EDGE_CURVE('',#40816,#40817,#4856,.T.);
#52428=EDGE_CURVE('',#40817,#40818,#33338,.T.);
#52429=EDGE_CURVE('',#40818,#40819,#4857,.T.);
#52430=EDGE_CURVE('',#40819,#40820,#22159,.T.);
#52431=EDGE_CURVE('',#40820,#40821,#33339,.T.);
#52432=EDGE_CURVE('',#40821,#40822,#22160,.T.);
#52433=EDGE_CURVE('',#40822,#40823,#4858,.T.);
#52434=EDGE_CURVE('',#40823,#40824,#33340,.T.);
#52435=EDGE_CURVE('',#40824,#40825,#4859,.T.);
#52436=EDGE_CURVE('',#40825,#40826,#22161,.T.);
#52437=EDGE_CURVE('',#40826,#40827,#33341,.T.);
#52438=EDGE_CURVE('',#40827,#40828,#22162,.T.);
#52439=EDGE_CURVE('',#40828,#40829,#4860,.T.);
#52440=EDGE_CURVE('',#40829,#40830,#33342,.T.);
#52441=EDGE_CURVE('',#40830,#40831,#4861,.T.);
#52442=EDGE_CURVE('',#40831,#40832,#22163,.T.);
#52443=EDGE_CURVE('',#40832,#40833,#33343,.T.);
#52444=EDGE_CURVE('',#40833,#40834,#22164,.T.);
#52445=EDGE_CURVE('',#40834,#40835,#4862,.T.);
#52446=EDGE_CURVE('',#40835,#40836,#33344,.T.);
#52447=EDGE_CURVE('',#40836,#40837,#4863,.T.);
#52448=EDGE_CURVE('',#40837,#40838,#22165,.T.);
#52449=EDGE_CURVE('',#40838,#40839,#33345,.T.);
#52450=EDGE_CURVE('',#40839,#40840,#22166,.T.);
#52451=EDGE_CURVE('',#40840,#40841,#4864,.T.);
#52452=EDGE_CURVE('',#40841,#40842,#33346,.T.);
#52453=EDGE_CURVE('',#40842,#40843,#4865,.T.);
#52454=EDGE_CURVE('',#40843,#40844,#22167,.T.);
#52455=EDGE_CURVE('',#40844,#40845,#33347,.T.);
#52456=EDGE_CURVE('',#40845,#40846,#22168,.T.);
#52457=EDGE_CURVE('',#40846,#40847,#4866,.T.);
#52458=EDGE_CURVE('',#40847,#40848,#33348,.T.);
#52459=EDGE_CURVE('',#40848,#40849,#4867,.T.);
#52460=EDGE_CURVE('',#40849,#40850,#22169,.T.);
#52461=EDGE_CURVE('',#40850,#40851,#33349,.T.);
#52462=EDGE_CURVE('',#40851,#40852,#22170,.T.);
#52463=EDGE_CURVE('',#40852,#40853,#4868,.T.);
#52464=EDGE_CURVE('',#40853,#40854,#33350,.T.);
#52465=EDGE_CURVE('',#40854,#40855,#4869,.T.);
#52466=EDGE_CURVE('',#40855,#40856,#22171,.T.);
#52467=EDGE_CURVE('',#40856,#40857,#33351,.T.);
#52468=EDGE_CURVE('',#40857,#40858,#22172,.T.);
#52469=EDGE_CURVE('',#40858,#40859,#4870,.T.);
#52470=EDGE_CURVE('',#40859,#40860,#33352,.T.);
#52471=EDGE_CURVE('',#40860,#40861,#4871,.T.);
#52472=EDGE_CURVE('',#40861,#40862,#22173,.T.);
#52473=EDGE_CURVE('',#40862,#40863,#33353,.T.);
#52474=EDGE_CURVE('',#40863,#40864,#22174,.T.);
#52475=EDGE_CURVE('',#40864,#40865,#4872,.T.);
#52476=EDGE_CURVE('',#40865,#40866,#33354,.T.);
#52477=EDGE_CURVE('',#40866,#40867,#4873,.T.);
#52478=EDGE_CURVE('',#40867,#40868,#22175,.T.);
#52479=EDGE_CURVE('',#40868,#40869,#33355,.T.);
#52480=EDGE_CURVE('',#40869,#40870,#22176,.T.);
#52481=EDGE_CURVE('',#40870,#40871,#4874,.T.);
#52482=EDGE_CURVE('',#40871,#40872,#33356,.T.);
#52483=EDGE_CURVE('',#40872,#40873,#4875,.T.);
#52484=EDGE_CURVE('',#40873,#40874,#22177,.T.);
#52485=EDGE_CURVE('',#40874,#40875,#33357,.T.);
#52486=EDGE_CURVE('',#40875,#40876,#22178,.T.);
#52487=EDGE_CURVE('',#40876,#40877,#4876,.T.);
#52488=EDGE_CURVE('',#40877,#40878,#33358,.T.);
#52489=EDGE_CURVE('',#40878,#40879,#4877,.T.);
#52490=EDGE_CURVE('',#40879,#40880,#22179,.T.);
#52491=EDGE_CURVE('',#40880,#40881,#33359,.T.);
#52492=EDGE_CURVE('',#40881,#40882,#22180,.T.);
#52493=EDGE_CURVE('',#40882,#40883,#4878,.T.);
#52494=EDGE_CURVE('',#40883,#40884,#33360,.T.);
#52495=EDGE_CURVE('',#40884,#40885,#4879,.T.);
#52496=EDGE_CURVE('',#40885,#40886,#22181,.T.);
#52497=EDGE_CURVE('',#40886,#40887,#33361,.T.);
#52498=EDGE_CURVE('',#40887,#40888,#22182,.T.);
#52499=EDGE_CURVE('',#40888,#40889,#4880,.T.);
#52500=EDGE_CURVE('',#40889,#40890,#33362,.T.);
#52501=EDGE_CURVE('',#40890,#40891,#4881,.T.);
#52502=EDGE_CURVE('',#40891,#40892,#22183,.T.);
#52503=EDGE_CURVE('',#40892,#40893,#33363,.T.);
#52504=EDGE_CURVE('',#40893,#40894,#22184,.T.);
#52505=EDGE_CURVE('',#40894,#40895,#4882,.T.);
#52506=EDGE_CURVE('',#40895,#40896,#33364,.T.);
#52507=EDGE_CURVE('',#40896,#40897,#4883,.T.);
#52508=EDGE_CURVE('',#40897,#40898,#22185,.T.);
#52509=EDGE_CURVE('',#40898,#40899,#33365,.T.);
#52510=EDGE_CURVE('',#40899,#40900,#22186,.T.);
#52511=EDGE_CURVE('',#40900,#40901,#4884,.T.);
#52512=EDGE_CURVE('',#40901,#40902,#33366,.T.);
#52513=EDGE_CURVE('',#40902,#40903,#4885,.T.);
#52514=EDGE_CURVE('',#40903,#40904,#22187,.T.);
#52515=EDGE_CURVE('',#40904,#40905,#33367,.T.);
#52516=EDGE_CURVE('',#40905,#40906,#22188,.T.);
#52517=EDGE_CURVE('',#40906,#40907,#4886,.T.);
#52518=EDGE_CURVE('',#40907,#40908,#33368,.T.);
#52519=EDGE_CURVE('',#40908,#40909,#4887,.T.);
#52520=EDGE_CURVE('',#40909,#40910,#22189,.T.);
#52521=EDGE_CURVE('',#40910,#40911,#33369,.T.);
#52522=EDGE_CURVE('',#40911,#40912,#22190,.T.);
#52523=EDGE_CURVE('',#40912,#40913,#4888,.T.);
#52524=EDGE_CURVE('',#40913,#40914,#33370,.T.);
#52525=EDGE_CURVE('',#40914,#40915,#4889,.T.);
#52526=EDGE_CURVE('',#40915,#40916,#22191,.T.);
#52527=EDGE_CURVE('',#40916,#40917,#33371,.T.);
#52528=EDGE_CURVE('',#40917,#40918,#22192,.T.);
#52529=EDGE_CURVE('',#40918,#40919,#4890,.T.);
#52530=EDGE_CURVE('',#40919,#40920,#33372,.T.);
#52531=EDGE_CURVE('',#40920,#40921,#4891,.T.);
#52532=EDGE_CURVE('',#40921,#40922,#22193,.T.);
#52533=EDGE_CURVE('',#40922,#40923,#33373,.T.);
#52534=EDGE_CURVE('',#40923,#40924,#22194,.T.);
#52535=EDGE_CURVE('',#40924,#40925,#4892,.T.);
#52536=EDGE_CURVE('',#40925,#40926,#33374,.T.);
#52537=EDGE_CURVE('',#40926,#40927,#4893,.T.);
#52538=EDGE_CURVE('',#40927,#40928,#22195,.T.);
#52539=EDGE_CURVE('',#40928,#40929,#33375,.T.);
#52540=EDGE_CURVE('',#40929,#40930,#22196,.T.);
#52541=EDGE_CURVE('',#40930,#40931,#4894,.T.);
#52542=EDGE_CURVE('',#40931,#40932,#33376,.T.);
#52543=EDGE_CURVE('',#40932,#40933,#4895,.T.);
#52544=EDGE_CURVE('',#40933,#40934,#22197,.T.);
#52545=EDGE_CURVE('',#40934,#40935,#33377,.T.);
#52546=EDGE_CURVE('',#40935,#40936,#22198,.T.);
#52547=EDGE_CURVE('',#40936,#40937,#4896,.T.);
#52548=EDGE_CURVE('',#40937,#40938,#33378,.T.);
#52549=EDGE_CURVE('',#40938,#40939,#4897,.T.);
#52550=EDGE_CURVE('',#40939,#40940,#22199,.T.);
#52551=EDGE_CURVE('',#40940,#40941,#33379,.T.);
#52552=EDGE_CURVE('',#40941,#40942,#22200,.T.);
#52553=EDGE_CURVE('',#40942,#40943,#4898,.T.);
#52554=EDGE_CURVE('',#40943,#40944,#33380,.T.);
#52555=EDGE_CURVE('',#40944,#40945,#4899,.T.);
#52556=EDGE_CURVE('',#40945,#40946,#22201,.T.);
#52557=EDGE_CURVE('',#40946,#40947,#33381,.T.);
#52558=EDGE_CURVE('',#40947,#40948,#22202,.T.);
#52559=EDGE_CURVE('',#40948,#40949,#4900,.T.);
#52560=EDGE_CURVE('',#40949,#40950,#33382,.T.);
#52561=EDGE_CURVE('',#40950,#40951,#4901,.T.);
#52562=EDGE_CURVE('',#40951,#40952,#22203,.T.);
#52563=EDGE_CURVE('',#40952,#40953,#33383,.T.);
#52564=EDGE_CURVE('',#40953,#40954,#22204,.T.);
#52565=EDGE_CURVE('',#40954,#40955,#4902,.T.);
#52566=EDGE_CURVE('',#40955,#40956,#33384,.T.);
#52567=EDGE_CURVE('',#40956,#40957,#4903,.T.);
#52568=EDGE_CURVE('',#40957,#40958,#22205,.T.);
#52569=EDGE_CURVE('',#40958,#40959,#33385,.T.);
#52570=EDGE_CURVE('',#40959,#40960,#22206,.T.);
#52571=EDGE_CURVE('',#40960,#40961,#4904,.T.);
#52572=EDGE_CURVE('',#40961,#40962,#33386,.T.);
#52573=EDGE_CURVE('',#40962,#40963,#4905,.T.);
#52574=EDGE_CURVE('',#40963,#40964,#22207,.T.);
#52575=EDGE_CURVE('',#40964,#40965,#33387,.T.);
#52576=EDGE_CURVE('',#40965,#40966,#22208,.T.);
#52577=EDGE_CURVE('',#40966,#40967,#4906,.T.);
#52578=EDGE_CURVE('',#40967,#40968,#33388,.T.);
#52579=EDGE_CURVE('',#40968,#40969,#4907,.T.);
#52580=EDGE_CURVE('',#40969,#40970,#22209,.T.);
#52581=EDGE_CURVE('',#40970,#40971,#33389,.T.);
#52582=EDGE_CURVE('',#40971,#40972,#22210,.T.);
#52583=EDGE_CURVE('',#40972,#40973,#4908,.T.);
#52584=EDGE_CURVE('',#40973,#40974,#33390,.T.);
#52585=EDGE_CURVE('',#40974,#40975,#4909,.T.);
#52586=EDGE_CURVE('',#40975,#40976,#22211,.T.);
#52587=EDGE_CURVE('',#40976,#40977,#33391,.T.);
#52588=EDGE_CURVE('',#40977,#40978,#22212,.T.);
#52589=EDGE_CURVE('',#40978,#40979,#4910,.T.);
#52590=EDGE_CURVE('',#40979,#40980,#33392,.T.);
#52591=EDGE_CURVE('',#40980,#40981,#4911,.T.);
#52592=EDGE_CURVE('',#40981,#40982,#22213,.T.);
#52593=EDGE_CURVE('',#40982,#40983,#33393,.T.);
#52594=EDGE_CURVE('',#40983,#40984,#22214,.T.);
#52595=EDGE_CURVE('',#40984,#40985,#4912,.T.);
#52596=EDGE_CURVE('',#40985,#40986,#33394,.T.);
#52597=EDGE_CURVE('',#40986,#40987,#4913,.T.);
#52598=EDGE_CURVE('',#40987,#40988,#22215,.T.);
#52599=EDGE_CURVE('',#40988,#40989,#33395,.T.);
#52600=EDGE_CURVE('',#40989,#40990,#22216,.T.);
#52601=EDGE_CURVE('',#40990,#40991,#4914,.T.);
#52602=EDGE_CURVE('',#40991,#40992,#33396,.T.);
#52603=EDGE_CURVE('',#40992,#40448,#22217,.T.);
#52604=EDGE_CURVE('',#40992,#40993,#33397,.T.);
#52605=EDGE_CURVE('',#40993,#40994,#4915,.T.);
#52606=EDGE_CURVE('',#40994,#40995,#22218,.T.);
#52607=EDGE_CURVE('',#40995,#40996,#33398,.T.);
#52608=EDGE_CURVE('',#40996,#40997,#22219,.T.);
#52609=EDGE_CURVE('',#40997,#40998,#4916,.T.);
#52610=EDGE_CURVE('',#40998,#40999,#33399,.T.);
#52611=EDGE_CURVE('',#40999,#41000,#4917,.T.);
#52612=EDGE_CURVE('',#41000,#41001,#22220,.T.);
#52613=EDGE_CURVE('',#41001,#41002,#33400,.T.);
#52614=EDGE_CURVE('',#41002,#41003,#22221,.T.);
#52615=EDGE_CURVE('',#41003,#41004,#4918,.T.);
#52616=EDGE_CURVE('',#41004,#41005,#33401,.T.);
#52617=EDGE_CURVE('',#41005,#41006,#4919,.T.);
#52618=EDGE_CURVE('',#41006,#41007,#22222,.T.);
#52619=EDGE_CURVE('',#41007,#41008,#33402,.T.);
#52620=EDGE_CURVE('',#41008,#41009,#22223,.T.);
#52621=EDGE_CURVE('',#41009,#41010,#4920,.T.);
#52622=EDGE_CURVE('',#41010,#41011,#33403,.T.);
#52623=EDGE_CURVE('',#41011,#41012,#4921,.T.);
#52624=EDGE_CURVE('',#41012,#41013,#22224,.T.);
#52625=EDGE_CURVE('',#41013,#41014,#33404,.T.);
#52626=EDGE_CURVE('',#41014,#41015,#22225,.T.);
#52627=EDGE_CURVE('',#41015,#41016,#4922,.T.);
#52628=EDGE_CURVE('',#41016,#41017,#33405,.T.);
#52629=EDGE_CURVE('',#41017,#41018,#4923,.T.);
#52630=EDGE_CURVE('',#41018,#41019,#22226,.T.);
#52631=EDGE_CURVE('',#41019,#41020,#33406,.T.);
#52632=EDGE_CURVE('',#41020,#41021,#22227,.T.);
#52633=EDGE_CURVE('',#41021,#41022,#4924,.T.);
#52634=EDGE_CURVE('',#41022,#41023,#33407,.T.);
#52635=EDGE_CURVE('',#41023,#41024,#4925,.T.);
#52636=EDGE_CURVE('',#41024,#41025,#22228,.T.);
#52637=EDGE_CURVE('',#41025,#41026,#33408,.T.);
#52638=EDGE_CURVE('',#41026,#41027,#22229,.T.);
#52639=EDGE_CURVE('',#41027,#41028,#4926,.T.);
#52640=EDGE_CURVE('',#41028,#41029,#33409,.T.);
#52641=EDGE_CURVE('',#41029,#41030,#4927,.T.);
#52642=EDGE_CURVE('',#41030,#41031,#22230,.T.);
#52643=EDGE_CURVE('',#41031,#41032,#33410,.T.);
#52644=EDGE_CURVE('',#41032,#41033,#22231,.T.);
#52645=EDGE_CURVE('',#41033,#41034,#4928,.T.);
#52646=EDGE_CURVE('',#41034,#41035,#33411,.T.);
#52647=EDGE_CURVE('',#41035,#41036,#4929,.T.);
#52648=EDGE_CURVE('',#41036,#41037,#22232,.T.);
#52649=EDGE_CURVE('',#41037,#41038,#33412,.T.);
#52650=EDGE_CURVE('',#41038,#41039,#22233,.T.);
#52651=EDGE_CURVE('',#41039,#41040,#4930,.T.);
#52652=EDGE_CURVE('',#41040,#41041,#33413,.T.);
#52653=EDGE_CURVE('',#41041,#41042,#4931,.T.);
#52654=EDGE_CURVE('',#41042,#41043,#22234,.T.);
#52655=EDGE_CURVE('',#41043,#41044,#33414,.T.);
#52656=EDGE_CURVE('',#41044,#41045,#22235,.T.);
#52657=EDGE_CURVE('',#41045,#41046,#4932,.T.);
#52658=EDGE_CURVE('',#41046,#41047,#33415,.T.);
#52659=EDGE_CURVE('',#41047,#41048,#4933,.T.);
#52660=EDGE_CURVE('',#41048,#41049,#22236,.T.);
#52661=EDGE_CURVE('',#41049,#41050,#33416,.T.);
#52662=EDGE_CURVE('',#41050,#41051,#22237,.T.);
#52663=EDGE_CURVE('',#41051,#41052,#4934,.T.);
#52664=EDGE_CURVE('',#41052,#41053,#33417,.T.);
#52665=EDGE_CURVE('',#41053,#41054,#4935,.T.);
#52666=EDGE_CURVE('',#41054,#41055,#22238,.T.);
#52667=EDGE_CURVE('',#41055,#41056,#33418,.T.);
#52668=EDGE_CURVE('',#41056,#41057,#22239,.T.);
#52669=EDGE_CURVE('',#41057,#41058,#4936,.T.);
#52670=EDGE_CURVE('',#41058,#41059,#33419,.T.);
#52671=EDGE_CURVE('',#41059,#41060,#4937,.T.);
#52672=EDGE_CURVE('',#41060,#41061,#22240,.T.);
#52673=EDGE_CURVE('',#41061,#41062,#33420,.T.);
#52674=EDGE_CURVE('',#41062,#41063,#22241,.T.);
#52675=EDGE_CURVE('',#41063,#41064,#4938,.T.);
#52676=EDGE_CURVE('',#41064,#41065,#33421,.T.);
#52677=EDGE_CURVE('',#41065,#41066,#4939,.T.);
#52678=EDGE_CURVE('',#41066,#41067,#22242,.T.);
#52679=EDGE_CURVE('',#41067,#41068,#33422,.T.);
#52680=EDGE_CURVE('',#41068,#41069,#22243,.T.);
#52681=EDGE_CURVE('',#41069,#41070,#4940,.T.);
#52682=EDGE_CURVE('',#41070,#41071,#33423,.T.);
#52683=EDGE_CURVE('',#41071,#41072,#4941,.T.);
#52684=EDGE_CURVE('',#41072,#41073,#22244,.T.);
#52685=EDGE_CURVE('',#41073,#41074,#33424,.T.);
#52686=EDGE_CURVE('',#41074,#41075,#22245,.T.);
#52687=EDGE_CURVE('',#41075,#41076,#4942,.T.);
#52688=EDGE_CURVE('',#41076,#41077,#33425,.T.);
#52689=EDGE_CURVE('',#41077,#41078,#4943,.T.);
#52690=EDGE_CURVE('',#41078,#41079,#22246,.T.);
#52691=EDGE_CURVE('',#41079,#41080,#33426,.T.);
#52692=EDGE_CURVE('',#41080,#41081,#22247,.T.);
#52693=EDGE_CURVE('',#41081,#40431,#4944,.T.);
#52694=EDGE_CURVE('',#40430,#41082,#4945,.T.);
#52695=EDGE_CURVE('',#41082,#41083,#22248,.T.);
#52696=EDGE_CURVE('',#41083,#41084,#33427,.T.);
#52697=EDGE_CURVE('',#41084,#41085,#22249,.T.);
#52698=EDGE_CURVE('',#41085,#41086,#4946,.T.);
#52699=EDGE_CURVE('',#41086,#41087,#33428,.T.);
#52700=EDGE_CURVE('',#41087,#41088,#4947,.T.);
#52701=EDGE_CURVE('',#41088,#41089,#22250,.T.);
#52702=EDGE_CURVE('',#41089,#41090,#33429,.T.);
#52703=EDGE_CURVE('',#41090,#41091,#22251,.T.);
#52704=EDGE_CURVE('',#41091,#41092,#4948,.T.);
#52705=EDGE_CURVE('',#41092,#41093,#33430,.T.);
#52706=EDGE_CURVE('',#41093,#41094,#4949,.T.);
#52707=EDGE_CURVE('',#41094,#41095,#22252,.T.);
#52708=EDGE_CURVE('',#41095,#41096,#33431,.T.);
#52709=EDGE_CURVE('',#41096,#41097,#22253,.T.);
#52710=EDGE_CURVE('',#41097,#41098,#4950,.T.);
#52711=EDGE_CURVE('',#41098,#41099,#33432,.T.);
#52712=EDGE_CURVE('',#41099,#41100,#4951,.T.);
#52713=EDGE_CURVE('',#41100,#41101,#22254,.T.);
#52714=EDGE_CURVE('',#41101,#41102,#33433,.T.);
#52715=EDGE_CURVE('',#41102,#41103,#22255,.T.);
#52716=EDGE_CURVE('',#41103,#41104,#4952,.T.);
#52717=EDGE_CURVE('',#41104,#41105,#33434,.T.);
#52718=EDGE_CURVE('',#41105,#41106,#4953,.T.);
#52719=EDGE_CURVE('',#41106,#41107,#22256,.T.);
#52720=EDGE_CURVE('',#41107,#41108,#33435,.T.);
#52721=EDGE_CURVE('',#41108,#41109,#22257,.T.);
#52722=EDGE_CURVE('',#41109,#41110,#4954,.T.);
#52723=EDGE_CURVE('',#41110,#41111,#33436,.T.);
#52724=EDGE_CURVE('',#41111,#41112,#4955,.T.);
#52725=EDGE_CURVE('',#41112,#41113,#22258,.T.);
#52726=EDGE_CURVE('',#41113,#41114,#33437,.T.);
#52727=EDGE_CURVE('',#41114,#41115,#22259,.T.);
#52728=EDGE_CURVE('',#41115,#41116,#4956,.T.);
#52729=EDGE_CURVE('',#41116,#41117,#33438,.T.);
#52730=EDGE_CURVE('',#41117,#41118,#4957,.T.);
#52731=EDGE_CURVE('',#41118,#41119,#22260,.T.);
#52732=EDGE_CURVE('',#41119,#41120,#33439,.T.);
#52733=EDGE_CURVE('',#41120,#41121,#22261,.T.);
#52734=EDGE_CURVE('',#41121,#41122,#4958,.T.);
#52735=EDGE_CURVE('',#41122,#41123,#33440,.T.);
#52736=EDGE_CURVE('',#41123,#41124,#4959,.T.);
#52737=EDGE_CURVE('',#41124,#41125,#22262,.T.);
#52738=EDGE_CURVE('',#41125,#41126,#33441,.T.);
#52739=EDGE_CURVE('',#41126,#41127,#22263,.T.);
#52740=EDGE_CURVE('',#41127,#41128,#4960,.T.);
#52741=EDGE_CURVE('',#41128,#41129,#33442,.T.);
#52742=EDGE_CURVE('',#41129,#41130,#4961,.T.);
#52743=EDGE_CURVE('',#41130,#41131,#22264,.T.);
#52744=EDGE_CURVE('',#41131,#41132,#33443,.T.);
#52745=EDGE_CURVE('',#41132,#41133,#22265,.T.);
#52746=EDGE_CURVE('',#41133,#41134,#4962,.T.);
#52747=EDGE_CURVE('',#41134,#41135,#33444,.T.);
#52748=EDGE_CURVE('',#41135,#41136,#4963,.T.);
#52749=EDGE_CURVE('',#41136,#41137,#22266,.T.);
#52750=EDGE_CURVE('',#41137,#41138,#33445,.T.);
#52751=EDGE_CURVE('',#41138,#41139,#22267,.T.);
#52752=EDGE_CURVE('',#41139,#41140,#4964,.T.);
#52753=EDGE_CURVE('',#41140,#41141,#33446,.T.);
#52754=EDGE_CURVE('',#41141,#41142,#4965,.T.);
#52755=EDGE_CURVE('',#41142,#41143,#22268,.T.);
#52756=EDGE_CURVE('',#41143,#41144,#33447,.T.);
#52757=EDGE_CURVE('',#41144,#41145,#22269,.T.);
#52758=EDGE_CURVE('',#41145,#41146,#4966,.T.);
#52759=EDGE_CURVE('',#41146,#41147,#33448,.T.);
#52760=EDGE_CURVE('',#41147,#41148,#4967,.T.);
#52761=EDGE_CURVE('',#41148,#41149,#22270,.T.);
#52762=EDGE_CURVE('',#41149,#41150,#33449,.T.);
#52763=EDGE_CURVE('',#41150,#41151,#22271,.T.);
#52764=EDGE_CURVE('',#41151,#41152,#4968,.T.);
#52765=EDGE_CURVE('',#41152,#41153,#33450,.T.);
#52766=EDGE_CURVE('',#41153,#41154,#4969,.T.);
#52767=EDGE_CURVE('',#41154,#41155,#22272,.T.);
#52768=EDGE_CURVE('',#41155,#41156,#33451,.T.);
#52769=EDGE_CURVE('',#41156,#41157,#22273,.T.);
#52770=EDGE_CURVE('',#41157,#41158,#4970,.T.);
#52771=EDGE_CURVE('',#41158,#41159,#33452,.T.);
#52772=EDGE_CURVE('',#41159,#41160,#4971,.T.);
#52773=EDGE_CURVE('',#41160,#41161,#22274,.T.);
#52774=EDGE_CURVE('',#41161,#41162,#33453,.T.);
#52775=EDGE_CURVE('',#41162,#41163,#22275,.T.);
#52776=EDGE_CURVE('',#41163,#41164,#4972,.T.);
#52777=EDGE_CURVE('',#41164,#41165,#33454,.T.);
#52778=EDGE_CURVE('',#41165,#41166,#4973,.T.);
#52779=EDGE_CURVE('',#41166,#41167,#22276,.T.);
#52780=EDGE_CURVE('',#41167,#41168,#33455,.T.);
#52781=EDGE_CURVE('',#41168,#41169,#22277,.T.);
#52782=EDGE_CURVE('',#41169,#40439,#4974,.T.);
#52783=EDGE_CURVE('',#41170,#41171,#33456,.T.);
#52784=EDGE_CURVE('',#41171,#40447,#22278,.T.);
#52785=EDGE_CURVE('',#41171,#41170,#33457,.T.);
#52786=EDGE_CURVE('',#41170,#41172,#22279,.T.);
#52787=EDGE_CURVE('',#41172,#41172,#33458,.T.);
#52788=EDGE_CURVE('',#41173,#41174,#33459,.T.);
#52789=EDGE_CURVE('',#41173,#41175,#22280,.T.);
#52790=EDGE_CURVE('',#41175,#41176,#33460,.T.);
#52791=EDGE_CURVE('',#41176,#41177,#22281,.T.);
#52792=EDGE_CURVE('',#41178,#41177,#33461,.T.);
#52793=EDGE_CURVE('',#41174,#41178,#33462,.T.);
#52794=EDGE_CURVE('',#41179,#41180,#33463,.T.);
#52795=EDGE_CURVE('',#41180,#41174,#22282,.T.);
#52796=EDGE_CURVE('',#41178,#41179,#22283,.T.);
#52797=EDGE_CURVE('',#41181,#41182,#33464,.T.);
#52798=EDGE_CURVE('',#41182,#41183,#22284,.T.);
#52799=EDGE_CURVE('',#41183,#41184,#33465,.T.);
#52800=EDGE_CURVE('',#41184,#41181,#22285,.T.);
#52801=EDGE_CURVE('',#41185,#41186,#33466,.T.);
#52802=EDGE_CURVE('',#41185,#41187,#22286,.T.);
#52803=EDGE_CURVE('',#41187,#41188,#33467,.T.);
#52804=EDGE_CURVE('',#41188,#41189,#22287,.T.);
#52805=EDGE_CURVE('',#41190,#41189,#33468,.T.);
#52806=EDGE_CURVE('',#41186,#41190,#33469,.T.);
#52807=EDGE_CURVE('',#41191,#41192,#33470,.T.);
#52808=EDGE_CURVE('',#41192,#41186,#22288,.T.);
#52809=EDGE_CURVE('',#41190,#41191,#22289,.T.);
#52810=EDGE_CURVE('',#41175,#40996,#33471,.T.);
#52811=EDGE_CURVE('',#40995,#41176,#33472,.T.);
#52812=EDGE_CURVE('',#40810,#41192,#1418,.T.);
#52813=EDGE_CURVE('',#41191,#40811,#1419,.T.);
#52814=EDGE_CURVE('',#41187,#41182,#1420,.T.);
#52815=EDGE_CURVE('',#41181,#41188,#1421,.T.);
#52816=EDGE_CURVE('',#41183,#41180,#1422,.T.);
#52817=EDGE_CURVE('',#41179,#41184,#1423,.T.);
#52818=EDGE_CURVE('',#41193,#41194,#33473,.T.);
#52819=EDGE_CURVE('',#41194,#41195,#22290,.T.);
#52820=EDGE_CURVE('',#41196,#41195,#33474,.T.);
#52821=EDGE_CURVE('',#41197,#41196,#33475,.T.);
#52822=EDGE_CURVE('',#41198,#41197,#33476,.T.);
#52823=EDGE_CURVE('',#41198,#41193,#22291,.T.);
#52824=EDGE_CURVE('',#41196,#41199,#22292,.T.);
#52825=EDGE_CURVE('',#41199,#41200,#33477,.T.);
#52826=EDGE_CURVE('',#41200,#41197,#22293,.T.);
#52827=EDGE_CURVE('',#41201,#41202,#33478,.T.);
#52828=EDGE_CURVE('',#41202,#41203,#22294,.T.);
#52829=EDGE_CURVE('',#41203,#41204,#33479,.T.);
#52830=EDGE_CURVE('',#41204,#41201,#22295,.T.);
#52831=EDGE_CURVE('',#41205,#41206,#33480,.T.);
#52832=EDGE_CURVE('',#41206,#41207,#22296,.T.);
#52833=EDGE_CURVE('',#41208,#41207,#33481,.T.);
#52834=EDGE_CURVE('',#41209,#41208,#33482,.T.);
#52835=EDGE_CURVE('',#41210,#41209,#33483,.T.);
#52836=EDGE_CURVE('',#41210,#41205,#22297,.T.);
#52837=EDGE_CURVE('',#41208,#41211,#22298,.T.);
#52838=EDGE_CURVE('',#41211,#41212,#33484,.T.);
#52839=EDGE_CURVE('',#41212,#41209,#22299,.T.);
#52840=EDGE_CURVE('',#41001,#41194,#33485,.T.);
#52841=EDGE_CURVE('',#41193,#41002,#33486,.T.);
#52842=EDGE_CURVE('',#41211,#40805,#1424,.T.);
#52843=EDGE_CURVE('',#40804,#41212,#1425,.T.);
#52844=EDGE_CURVE('',#41203,#41206,#1426,.T.);
#52845=EDGE_CURVE('',#41205,#41204,#1427,.T.);
#52846=EDGE_CURVE('',#41199,#41202,#1428,.T.);
#52847=EDGE_CURVE('',#41201,#41200,#1429,.T.);
#52848=EDGE_CURVE('',#41213,#41214,#33487,.T.);
#52849=EDGE_CURVE('',#41214,#41215,#22300,.T.);
#52850=EDGE_CURVE('',#41216,#41215,#33488,.T.);
#52851=EDGE_CURVE('',#41217,#41216,#33489,.T.);
#52852=EDGE_CURVE('',#41218,#41217,#33490,.T.);
#52853=EDGE_CURVE('',#41218,#41213,#22301,.T.);
#52854=EDGE_CURVE('',#41216,#41219,#22302,.T.);
#52855=EDGE_CURVE('',#41219,#41220,#33491,.T.);
#52856=EDGE_CURVE('',#41220,#41217,#22303,.T.);
#52857=EDGE_CURVE('',#41221,#41222,#33492,.T.);
#52858=EDGE_CURVE('',#41222,#41223,#22304,.T.);
#52859=EDGE_CURVE('',#41223,#41224,#33493,.T.);
#52860=EDGE_CURVE('',#41224,#41221,#22305,.T.);
#52861=EDGE_CURVE('',#41225,#41226,#33494,.T.);
#52862=EDGE_CURVE('',#41226,#41227,#22306,.T.);
#52863=EDGE_CURVE('',#41228,#41227,#33495,.T.);
#52864=EDGE_CURVE('',#41229,#41228,#33496,.T.);
#52865=EDGE_CURVE('',#41230,#41229,#33497,.T.);
#52866=EDGE_CURVE('',#41230,#41225,#22307,.T.);
#52867=EDGE_CURVE('',#41228,#41231,#22308,.T.);
#52868=EDGE_CURVE('',#41231,#41232,#33498,.T.);
#52869=EDGE_CURVE('',#41232,#41229,#22309,.T.);
#52870=EDGE_CURVE('',#41007,#41214,#33499,.T.);
#52871=EDGE_CURVE('',#41213,#41008,#33500,.T.);
#52872=EDGE_CURVE('',#41231,#40799,#1430,.T.);
#52873=EDGE_CURVE('',#40798,#41232,#1431,.T.);
#52874=EDGE_CURVE('',#41223,#41226,#1432,.T.);
#52875=EDGE_CURVE('',#41225,#41224,#1433,.T.);
#52876=EDGE_CURVE('',#41219,#41222,#1434,.T.);
#52877=EDGE_CURVE('',#41221,#41220,#1435,.T.);
#52878=EDGE_CURVE('',#41233,#41234,#33501,.T.);
#52879=EDGE_CURVE('',#41234,#41235,#22310,.T.);
#52880=EDGE_CURVE('',#41236,#41235,#33502,.T.);
#52881=EDGE_CURVE('',#41237,#41236,#33503,.T.);
#52882=EDGE_CURVE('',#41238,#41237,#33504,.T.);
#52883=EDGE_CURVE('',#41238,#41233,#22311,.T.);
#52884=EDGE_CURVE('',#41236,#41239,#22312,.T.);
#52885=EDGE_CURVE('',#41239,#41240,#33505,.T.);
#52886=EDGE_CURVE('',#41240,#41237,#22313,.T.);
#52887=EDGE_CURVE('',#41241,#41242,#33506,.T.);
#52888=EDGE_CURVE('',#41242,#41243,#22314,.T.);
#52889=EDGE_CURVE('',#41243,#41244,#33507,.T.);
#52890=EDGE_CURVE('',#41244,#41241,#22315,.T.);
#52891=EDGE_CURVE('',#41245,#41246,#33508,.T.);
#52892=EDGE_CURVE('',#41246,#41247,#22316,.T.);
#52893=EDGE_CURVE('',#41248,#41247,#33509,.T.);
#52894=EDGE_CURVE('',#41249,#41248,#33510,.T.);
#52895=EDGE_CURVE('',#41250,#41249,#33511,.T.);
#52896=EDGE_CURVE('',#41250,#41245,#22317,.T.);
#52897=EDGE_CURVE('',#41248,#41251,#22318,.T.);
#52898=EDGE_CURVE('',#41251,#41252,#33512,.T.);
#52899=EDGE_CURVE('',#41252,#41249,#22319,.T.);
#52900=EDGE_CURVE('',#41013,#41234,#33513,.T.);
#52901=EDGE_CURVE('',#41233,#41014,#33514,.T.);
#52902=EDGE_CURVE('',#41251,#40793,#1436,.T.);
#52903=EDGE_CURVE('',#40792,#41252,#1437,.T.);
#52904=EDGE_CURVE('',#41243,#41246,#1438,.T.);
#52905=EDGE_CURVE('',#41245,#41244,#1439,.T.);
#52906=EDGE_CURVE('',#41239,#41242,#1440,.T.);
#52907=EDGE_CURVE('',#41241,#41240,#1441,.T.);
#52908=EDGE_CURVE('',#41253,#41254,#33515,.T.);
#52909=EDGE_CURVE('',#41254,#41255,#22320,.T.);
#52910=EDGE_CURVE('',#41256,#41255,#33516,.T.);
#52911=EDGE_CURVE('',#41257,#41256,#33517,.T.);
#52912=EDGE_CURVE('',#41258,#41257,#33518,.T.);
#52913=EDGE_CURVE('',#41258,#41253,#22321,.T.);
#52914=EDGE_CURVE('',#41256,#41259,#22322,.T.);
#52915=EDGE_CURVE('',#41259,#41260,#33519,.T.);
#52916=EDGE_CURVE('',#41260,#41257,#22323,.T.);
#52917=EDGE_CURVE('',#41261,#41262,#33520,.T.);
#52918=EDGE_CURVE('',#41262,#41263,#22324,.T.);
#52919=EDGE_CURVE('',#41263,#41264,#33521,.T.);
#52920=EDGE_CURVE('',#41264,#41261,#22325,.T.);
#52921=EDGE_CURVE('',#41265,#41266,#33522,.T.);
#52922=EDGE_CURVE('',#41266,#41267,#22326,.T.);
#52923=EDGE_CURVE('',#41268,#41267,#33523,.T.);
#52924=EDGE_CURVE('',#41269,#41268,#33524,.T.);
#52925=EDGE_CURVE('',#41270,#41269,#33525,.T.);
#52926=EDGE_CURVE('',#41270,#41265,#22327,.T.);
#52927=EDGE_CURVE('',#41268,#41271,#22328,.T.);
#52928=EDGE_CURVE('',#41271,#41272,#33526,.T.);
#52929=EDGE_CURVE('',#41272,#41269,#22329,.T.);
#52930=EDGE_CURVE('',#41019,#41254,#33527,.T.);
#52931=EDGE_CURVE('',#41253,#41020,#33528,.T.);
#52932=EDGE_CURVE('',#41271,#40787,#1442,.T.);
#52933=EDGE_CURVE('',#40786,#41272,#1443,.T.);
#52934=EDGE_CURVE('',#41263,#41266,#1444,.T.);
#52935=EDGE_CURVE('',#41265,#41264,#1445,.T.);
#52936=EDGE_CURVE('',#41259,#41262,#1446,.T.);
#52937=EDGE_CURVE('',#41261,#41260,#1447,.T.);
#52938=EDGE_CURVE('',#41273,#41274,#33529,.T.);
#52939=EDGE_CURVE('',#41274,#41275,#22330,.T.);
#52940=EDGE_CURVE('',#41276,#41275,#33530,.T.);
#52941=EDGE_CURVE('',#41277,#41276,#33531,.T.);
#52942=EDGE_CURVE('',#41278,#41277,#33532,.T.);
#52943=EDGE_CURVE('',#41278,#41273,#22331,.T.);
#52944=EDGE_CURVE('',#41276,#41279,#22332,.T.);
#52945=EDGE_CURVE('',#41279,#41280,#33533,.T.);
#52946=EDGE_CURVE('',#41280,#41277,#22333,.T.);
#52947=EDGE_CURVE('',#41281,#41282,#33534,.T.);
#52948=EDGE_CURVE('',#41282,#41283,#22334,.T.);
#52949=EDGE_CURVE('',#41283,#41284,#33535,.T.);
#52950=EDGE_CURVE('',#41284,#41281,#22335,.T.);
#52951=EDGE_CURVE('',#41285,#41286,#33536,.T.);
#52952=EDGE_CURVE('',#41286,#41287,#22336,.T.);
#52953=EDGE_CURVE('',#41288,#41287,#33537,.T.);
#52954=EDGE_CURVE('',#41289,#41288,#33538,.T.);
#52955=EDGE_CURVE('',#41290,#41289,#33539,.T.);
#52956=EDGE_CURVE('',#41290,#41285,#22337,.T.);
#52957=EDGE_CURVE('',#41288,#41291,#22338,.T.);
#52958=EDGE_CURVE('',#41291,#41292,#33540,.T.);
#52959=EDGE_CURVE('',#41292,#41289,#22339,.T.);
#52960=EDGE_CURVE('',#41025,#41274,#33541,.T.);
#52961=EDGE_CURVE('',#41273,#41026,#33542,.T.);
#52962=EDGE_CURVE('',#41291,#40781,#1448,.T.);
#52963=EDGE_CURVE('',#40780,#41292,#1449,.T.);
#52964=EDGE_CURVE('',#41283,#41286,#1450,.T.);
#52965=EDGE_CURVE('',#41285,#41284,#1451,.T.);
#52966=EDGE_CURVE('',#41279,#41282,#1452,.T.);
#52967=EDGE_CURVE('',#41281,#41280,#1453,.T.);
#52968=EDGE_CURVE('',#41293,#41294,#33543,.T.);
#52969=EDGE_CURVE('',#41294,#41295,#22340,.T.);
#52970=EDGE_CURVE('',#41296,#41295,#33544,.T.);
#52971=EDGE_CURVE('',#41297,#41296,#33545,.T.);
#52972=EDGE_CURVE('',#41298,#41297,#33546,.T.);
#52973=EDGE_CURVE('',#41298,#41293,#22341,.T.);
#52974=EDGE_CURVE('',#41296,#41299,#22342,.T.);
#52975=EDGE_CURVE('',#41299,#41300,#33547,.T.);
#52976=EDGE_CURVE('',#41300,#41297,#22343,.T.);
#52977=EDGE_CURVE('',#41301,#41302,#33548,.T.);
#52978=EDGE_CURVE('',#41302,#41303,#22344,.T.);
#52979=EDGE_CURVE('',#41303,#41304,#33549,.T.);
#52980=EDGE_CURVE('',#41304,#41301,#22345,.T.);
#52981=EDGE_CURVE('',#41305,#41306,#33550,.T.);
#52982=EDGE_CURVE('',#41306,#41307,#22346,.T.);
#52983=EDGE_CURVE('',#41308,#41307,#33551,.T.);
#52984=EDGE_CURVE('',#41309,#41308,#33552,.T.);
#52985=EDGE_CURVE('',#41310,#41309,#33553,.T.);
#52986=EDGE_CURVE('',#41310,#41305,#22347,.T.);
#52987=EDGE_CURVE('',#41308,#41311,#22348,.T.);
#52988=EDGE_CURVE('',#41311,#41312,#33554,.T.);
#52989=EDGE_CURVE('',#41312,#41309,#22349,.T.);
#52990=EDGE_CURVE('',#41031,#41294,#33555,.T.);
#52991=EDGE_CURVE('',#41293,#41032,#33556,.T.);
#52992=EDGE_CURVE('',#41311,#40775,#1454,.T.);
#52993=EDGE_CURVE('',#40774,#41312,#1455,.T.);
#52994=EDGE_CURVE('',#41303,#41306,#1456,.T.);
#52995=EDGE_CURVE('',#41305,#41304,#1457,.T.);
#52996=EDGE_CURVE('',#41299,#41302,#1458,.T.);
#52997=EDGE_CURVE('',#41301,#41300,#1459,.T.);
#52998=EDGE_CURVE('',#41313,#41314,#33557,.T.);
#52999=EDGE_CURVE('',#41314,#41315,#22350,.T.);
#53000=EDGE_CURVE('',#41316,#41315,#33558,.T.);
#53001=EDGE_CURVE('',#41317,#41316,#33559,.T.);
#53002=EDGE_CURVE('',#41318,#41317,#33560,.T.);
#53003=EDGE_CURVE('',#41318,#41313,#22351,.T.);
#53004=EDGE_CURVE('',#41316,#41319,#22352,.T.);
#53005=EDGE_CURVE('',#41319,#41320,#33561,.T.);
#53006=EDGE_CURVE('',#41320,#41317,#22353,.T.);
#53007=EDGE_CURVE('',#41321,#41322,#33562,.T.);
#53008=EDGE_CURVE('',#41322,#41323,#22354,.T.);
#53009=EDGE_CURVE('',#41323,#41324,#33563,.T.);
#53010=EDGE_CURVE('',#41324,#41321,#22355,.T.);
#53011=EDGE_CURVE('',#41325,#41326,#33564,.T.);
#53012=EDGE_CURVE('',#41326,#41327,#22356,.T.);
#53013=EDGE_CURVE('',#41328,#41327,#33565,.T.);
#53014=EDGE_CURVE('',#41329,#41328,#33566,.T.);
#53015=EDGE_CURVE('',#41330,#41329,#33567,.T.);
#53016=EDGE_CURVE('',#41330,#41325,#22357,.T.);
#53017=EDGE_CURVE('',#41328,#41331,#22358,.T.);
#53018=EDGE_CURVE('',#41331,#41332,#33568,.T.);
#53019=EDGE_CURVE('',#41332,#41329,#22359,.T.);
#53020=EDGE_CURVE('',#41037,#41314,#33569,.T.);
#53021=EDGE_CURVE('',#41313,#41038,#33570,.T.);
#53022=EDGE_CURVE('',#41331,#40769,#1460,.T.);
#53023=EDGE_CURVE('',#40768,#41332,#1461,.T.);
#53024=EDGE_CURVE('',#41323,#41326,#1462,.T.);
#53025=EDGE_CURVE('',#41325,#41324,#1463,.T.);
#53026=EDGE_CURVE('',#41319,#41322,#1464,.T.);
#53027=EDGE_CURVE('',#41321,#41320,#1465,.T.);
#53028=EDGE_CURVE('',#41333,#41334,#33571,.T.);
#53029=EDGE_CURVE('',#41334,#41335,#22360,.T.);
#53030=EDGE_CURVE('',#41336,#41335,#33572,.T.);
#53031=EDGE_CURVE('',#41337,#41336,#33573,.T.);
#53032=EDGE_CURVE('',#41338,#41337,#33574,.T.);
#53033=EDGE_CURVE('',#41338,#41333,#22361,.T.);
#53034=EDGE_CURVE('',#41336,#41339,#22362,.T.);
#53035=EDGE_CURVE('',#41339,#41340,#33575,.T.);
#53036=EDGE_CURVE('',#41340,#41337,#22363,.T.);
#53037=EDGE_CURVE('',#41341,#41342,#33576,.T.);
#53038=EDGE_CURVE('',#41342,#41343,#22364,.T.);
#53039=EDGE_CURVE('',#41343,#41344,#33577,.T.);
#53040=EDGE_CURVE('',#41344,#41341,#22365,.T.);
#53041=EDGE_CURVE('',#41345,#41346,#33578,.T.);
#53042=EDGE_CURVE('',#41346,#41347,#22366,.T.);
#53043=EDGE_CURVE('',#41348,#41347,#33579,.T.);
#53044=EDGE_CURVE('',#41349,#41348,#33580,.T.);
#53045=EDGE_CURVE('',#41350,#41349,#33581,.T.);
#53046=EDGE_CURVE('',#41350,#41345,#22367,.T.);
#53047=EDGE_CURVE('',#41348,#41351,#22368,.T.);
#53048=EDGE_CURVE('',#41351,#41352,#33582,.T.);
#53049=EDGE_CURVE('',#41352,#41349,#22369,.T.);
#53050=EDGE_CURVE('',#41043,#41334,#33583,.T.);
#53051=EDGE_CURVE('',#41333,#41044,#33584,.T.);
#53052=EDGE_CURVE('',#41351,#40763,#1466,.T.);
#53053=EDGE_CURVE('',#40762,#41352,#1467,.T.);
#53054=EDGE_CURVE('',#41343,#41346,#1468,.T.);
#53055=EDGE_CURVE('',#41345,#41344,#1469,.T.);
#53056=EDGE_CURVE('',#41339,#41342,#1470,.T.);
#53057=EDGE_CURVE('',#41341,#41340,#1471,.T.);
#53058=EDGE_CURVE('',#41353,#41354,#33585,.T.);
#53059=EDGE_CURVE('',#41354,#41355,#22370,.T.);
#53060=EDGE_CURVE('',#41356,#41355,#33586,.T.);
#53061=EDGE_CURVE('',#41357,#41356,#33587,.T.);
#53062=EDGE_CURVE('',#41358,#41357,#33588,.T.);
#53063=EDGE_CURVE('',#41358,#41353,#22371,.T.);
#53064=EDGE_CURVE('',#41356,#41359,#22372,.T.);
#53065=EDGE_CURVE('',#41359,#41360,#33589,.T.);
#53066=EDGE_CURVE('',#41360,#41357,#22373,.T.);
#53067=EDGE_CURVE('',#41361,#41362,#33590,.T.);
#53068=EDGE_CURVE('',#41362,#41363,#22374,.T.);
#53069=EDGE_CURVE('',#41363,#41364,#33591,.T.);
#53070=EDGE_CURVE('',#41364,#41361,#22375,.T.);
#53071=EDGE_CURVE('',#41365,#41366,#33592,.T.);
#53072=EDGE_CURVE('',#41366,#41367,#22376,.T.);
#53073=EDGE_CURVE('',#41368,#41367,#33593,.T.);
#53074=EDGE_CURVE('',#41369,#41368,#33594,.T.);
#53075=EDGE_CURVE('',#41370,#41369,#33595,.T.);
#53076=EDGE_CURVE('',#41370,#41365,#22377,.T.);
#53077=EDGE_CURVE('',#41368,#41371,#22378,.T.);
#53078=EDGE_CURVE('',#41371,#41372,#33596,.T.);
#53079=EDGE_CURVE('',#41372,#41369,#22379,.T.);
#53080=EDGE_CURVE('',#41049,#41354,#33597,.T.);
#53081=EDGE_CURVE('',#41353,#41050,#33598,.T.);
#53082=EDGE_CURVE('',#41371,#40757,#1472,.T.);
#53083=EDGE_CURVE('',#40756,#41372,#1473,.T.);
#53084=EDGE_CURVE('',#41363,#41366,#1474,.T.);
#53085=EDGE_CURVE('',#41365,#41364,#1475,.T.);
#53086=EDGE_CURVE('',#41359,#41362,#1476,.T.);
#53087=EDGE_CURVE('',#41361,#41360,#1477,.T.);
#53088=EDGE_CURVE('',#41373,#41374,#33599,.T.);
#53089=EDGE_CURVE('',#41374,#41375,#22380,.T.);
#53090=EDGE_CURVE('',#41376,#41375,#33600,.T.);
#53091=EDGE_CURVE('',#41377,#41376,#33601,.T.);
#53092=EDGE_CURVE('',#41378,#41377,#33602,.T.);
#53093=EDGE_CURVE('',#41378,#41373,#22381,.T.);
#53094=EDGE_CURVE('',#41376,#41379,#22382,.T.);
#53095=EDGE_CURVE('',#41379,#41380,#33603,.T.);
#53096=EDGE_CURVE('',#41380,#41377,#22383,.T.);
#53097=EDGE_CURVE('',#41381,#41382,#33604,.T.);
#53098=EDGE_CURVE('',#41382,#41383,#22384,.T.);
#53099=EDGE_CURVE('',#41383,#41384,#33605,.T.);
#53100=EDGE_CURVE('',#41384,#41381,#22385,.T.);
#53101=EDGE_CURVE('',#41385,#41386,#33606,.T.);
#53102=EDGE_CURVE('',#41386,#41387,#22386,.T.);
#53103=EDGE_CURVE('',#41388,#41387,#33607,.T.);
#53104=EDGE_CURVE('',#41389,#41388,#33608,.T.);
#53105=EDGE_CURVE('',#41390,#41389,#33609,.T.);
#53106=EDGE_CURVE('',#41390,#41385,#22387,.T.);
#53107=EDGE_CURVE('',#41388,#41391,#22388,.T.);
#53108=EDGE_CURVE('',#41391,#41392,#33610,.T.);
#53109=EDGE_CURVE('',#41392,#41389,#22389,.T.);
#53110=EDGE_CURVE('',#41055,#41374,#33611,.T.);
#53111=EDGE_CURVE('',#41373,#41056,#33612,.T.);
#53112=EDGE_CURVE('',#41391,#40751,#1478,.T.);
#53113=EDGE_CURVE('',#40750,#41392,#1479,.T.);
#53114=EDGE_CURVE('',#41383,#41386,#1480,.T.);
#53115=EDGE_CURVE('',#41385,#41384,#1481,.T.);
#53116=EDGE_CURVE('',#41379,#41382,#1482,.T.);
#53117=EDGE_CURVE('',#41381,#41380,#1483,.T.);
#53118=EDGE_CURVE('',#41393,#41394,#33613,.T.);
#53119=EDGE_CURVE('',#41394,#41395,#22390,.T.);
#53120=EDGE_CURVE('',#41396,#41395,#33614,.T.);
#53121=EDGE_CURVE('',#41397,#41396,#33615,.T.);
#53122=EDGE_CURVE('',#41398,#41397,#33616,.T.);
#53123=EDGE_CURVE('',#41398,#41393,#22391,.T.);
#53124=EDGE_CURVE('',#41396,#41399,#22392,.T.);
#53125=EDGE_CURVE('',#41399,#41400,#33617,.T.);
#53126=EDGE_CURVE('',#41400,#41397,#22393,.T.);
#53127=EDGE_CURVE('',#41401,#41402,#33618,.T.);
#53128=EDGE_CURVE('',#41402,#41403,#22394,.T.);
#53129=EDGE_CURVE('',#41403,#41404,#33619,.T.);
#53130=EDGE_CURVE('',#41404,#41401,#22395,.T.);
#53131=EDGE_CURVE('',#41405,#41406,#33620,.T.);
#53132=EDGE_CURVE('',#41406,#41407,#22396,.T.);
#53133=EDGE_CURVE('',#41408,#41407,#33621,.T.);
#53134=EDGE_CURVE('',#41409,#41408,#33622,.T.);
#53135=EDGE_CURVE('',#41410,#41409,#33623,.T.);
#53136=EDGE_CURVE('',#41410,#41405,#22397,.T.);
#53137=EDGE_CURVE('',#41408,#41411,#22398,.T.);
#53138=EDGE_CURVE('',#41411,#41412,#33624,.T.);
#53139=EDGE_CURVE('',#41412,#41409,#22399,.T.);
#53140=EDGE_CURVE('',#41061,#41394,#33625,.T.);
#53141=EDGE_CURVE('',#41393,#41062,#33626,.T.);
#53142=EDGE_CURVE('',#41411,#40745,#1484,.T.);
#53143=EDGE_CURVE('',#40744,#41412,#1485,.T.);
#53144=EDGE_CURVE('',#41403,#41406,#1486,.T.);
#53145=EDGE_CURVE('',#41405,#41404,#1487,.T.);
#53146=EDGE_CURVE('',#41399,#41402,#1488,.T.);
#53147=EDGE_CURVE('',#41401,#41400,#1489,.T.);
#53148=EDGE_CURVE('',#41413,#41414,#33627,.T.);
#53149=EDGE_CURVE('',#41414,#41415,#22400,.T.);
#53150=EDGE_CURVE('',#41416,#41415,#33628,.T.);
#53151=EDGE_CURVE('',#41417,#41416,#33629,.T.);
#53152=EDGE_CURVE('',#41418,#41417,#33630,.T.);
#53153=EDGE_CURVE('',#41418,#41413,#22401,.T.);
#53154=EDGE_CURVE('',#41416,#41419,#22402,.T.);
#53155=EDGE_CURVE('',#41419,#41420,#33631,.T.);
#53156=EDGE_CURVE('',#41420,#41417,#22403,.T.);
#53157=EDGE_CURVE('',#41421,#41422,#33632,.T.);
#53158=EDGE_CURVE('',#41422,#41423,#22404,.T.);
#53159=EDGE_CURVE('',#41423,#41424,#33633,.T.);
#53160=EDGE_CURVE('',#41424,#41421,#22405,.T.);
#53161=EDGE_CURVE('',#41425,#41426,#33634,.T.);
#53162=EDGE_CURVE('',#41426,#41427,#22406,.T.);
#53163=EDGE_CURVE('',#41428,#41427,#33635,.T.);
#53164=EDGE_CURVE('',#41429,#41428,#33636,.T.);
#53165=EDGE_CURVE('',#41430,#41429,#33637,.T.);
#53166=EDGE_CURVE('',#41430,#41425,#22407,.T.);
#53167=EDGE_CURVE('',#41428,#41431,#22408,.T.);
#53168=EDGE_CURVE('',#41431,#41432,#33638,.T.);
#53169=EDGE_CURVE('',#41432,#41429,#22409,.T.);
#53170=EDGE_CURVE('',#41067,#41414,#33639,.T.);
#53171=EDGE_CURVE('',#41413,#41068,#33640,.T.);
#53172=EDGE_CURVE('',#41431,#40739,#1490,.T.);
#53173=EDGE_CURVE('',#40738,#41432,#1491,.T.);
#53174=EDGE_CURVE('',#41423,#41426,#1492,.T.);
#53175=EDGE_CURVE('',#41425,#41424,#1493,.T.);
#53176=EDGE_CURVE('',#41419,#41422,#1494,.T.);
#53177=EDGE_CURVE('',#41421,#41420,#1495,.T.);
#53178=EDGE_CURVE('',#41433,#41434,#33641,.T.);
#53179=EDGE_CURVE('',#41434,#41435,#22410,.T.);
#53180=EDGE_CURVE('',#41436,#41435,#33642,.T.);
#53181=EDGE_CURVE('',#41437,#41436,#33643,.T.);
#53182=EDGE_CURVE('',#41438,#41437,#33644,.T.);
#53183=EDGE_CURVE('',#41438,#41433,#22411,.T.);
#53184=EDGE_CURVE('',#41436,#41439,#22412,.T.);
#53185=EDGE_CURVE('',#41439,#41440,#33645,.T.);
#53186=EDGE_CURVE('',#41440,#41437,#22413,.T.);
#53187=EDGE_CURVE('',#41441,#41442,#33646,.T.);
#53188=EDGE_CURVE('',#41442,#41443,#22414,.T.);
#53189=EDGE_CURVE('',#41443,#41444,#33647,.T.);
#53190=EDGE_CURVE('',#41444,#41441,#22415,.T.);
#53191=EDGE_CURVE('',#41445,#41446,#33648,.T.);
#53192=EDGE_CURVE('',#41446,#41447,#22416,.T.);
#53193=EDGE_CURVE('',#41448,#41447,#33649,.T.);
#53194=EDGE_CURVE('',#41449,#41448,#33650,.T.);
#53195=EDGE_CURVE('',#41450,#41449,#33651,.T.);
#53196=EDGE_CURVE('',#41450,#41445,#22417,.T.);
#53197=EDGE_CURVE('',#41448,#41451,#22418,.T.);
#53198=EDGE_CURVE('',#41451,#41452,#33652,.T.);
#53199=EDGE_CURVE('',#41452,#41449,#22419,.T.);
#53200=EDGE_CURVE('',#41073,#41434,#33653,.T.);
#53201=EDGE_CURVE('',#41433,#41074,#33654,.T.);
#53202=EDGE_CURVE('',#41451,#40733,#1496,.T.);
#53203=EDGE_CURVE('',#40732,#41452,#1497,.T.);
#53204=EDGE_CURVE('',#41443,#41446,#1498,.T.);
#53205=EDGE_CURVE('',#41445,#41444,#1499,.T.);
#53206=EDGE_CURVE('',#41439,#41442,#1500,.T.);
#53207=EDGE_CURVE('',#41441,#41440,#1501,.T.);
#53208=EDGE_CURVE('',#41453,#41454,#33655,.T.);
#53209=EDGE_CURVE('',#41454,#41455,#22420,.T.);
#53210=EDGE_CURVE('',#41456,#41455,#33656,.T.);
#53211=EDGE_CURVE('',#41457,#41456,#33657,.T.);
#53212=EDGE_CURVE('',#41458,#41457,#33658,.T.);
#53213=EDGE_CURVE('',#41458,#41453,#22421,.T.);
#53214=EDGE_CURVE('',#41456,#41459,#22422,.T.);
#53215=EDGE_CURVE('',#41459,#41460,#33659,.T.);
#53216=EDGE_CURVE('',#41460,#41457,#22423,.T.);
#53217=EDGE_CURVE('',#41461,#41462,#33660,.T.);
#53218=EDGE_CURVE('',#41462,#41463,#22424,.T.);
#53219=EDGE_CURVE('',#41463,#41464,#33661,.T.);
#53220=EDGE_CURVE('',#41464,#41461,#22425,.T.);
#53221=EDGE_CURVE('',#41465,#41466,#33662,.T.);
#53222=EDGE_CURVE('',#41466,#41467,#22426,.T.);
#53223=EDGE_CURVE('',#41468,#41467,#33663,.T.);
#53224=EDGE_CURVE('',#41469,#41468,#33664,.T.);
#53225=EDGE_CURVE('',#41470,#41469,#33665,.T.);
#53226=EDGE_CURVE('',#41470,#41465,#22427,.T.);
#53227=EDGE_CURVE('',#41468,#41471,#22428,.T.);
#53228=EDGE_CURVE('',#41471,#41472,#33666,.T.);
#53229=EDGE_CURVE('',#41472,#41469,#22429,.T.);
#53230=EDGE_CURVE('',#41079,#41454,#33667,.T.);
#53231=EDGE_CURVE('',#41453,#41080,#33668,.T.);
#53232=EDGE_CURVE('',#41471,#40727,#1502,.T.);
#53233=EDGE_CURVE('',#40726,#41472,#1503,.T.);
#53234=EDGE_CURVE('',#41463,#41466,#1504,.T.);
#53235=EDGE_CURVE('',#41465,#41464,#1505,.T.);
#53236=EDGE_CURVE('',#41459,#41462,#1506,.T.);
#53237=EDGE_CURVE('',#41461,#41460,#1507,.T.);
#53238=EDGE_CURVE('',#41473,#41474,#33669,.T.);
#53239=EDGE_CURVE('',#41474,#41475,#22430,.T.);
#53240=EDGE_CURVE('',#41476,#41475,#33670,.T.);
#53241=EDGE_CURVE('',#41477,#41476,#33671,.T.);
#53242=EDGE_CURVE('',#41478,#41477,#33672,.T.);
#53243=EDGE_CURVE('',#41478,#41473,#22431,.T.);
#53244=EDGE_CURVE('',#41476,#41479,#22432,.T.);
#53245=EDGE_CURVE('',#41479,#41480,#33673,.T.);
#53246=EDGE_CURVE('',#41480,#41477,#22433,.T.);
#53247=EDGE_CURVE('',#41481,#41482,#33674,.T.);
#53248=EDGE_CURVE('',#41482,#41483,#22434,.T.);
#53249=EDGE_CURVE('',#41483,#41484,#33675,.T.);
#53250=EDGE_CURVE('',#41484,#41481,#22435,.T.);
#53251=EDGE_CURVE('',#41485,#41486,#33676,.T.);
#53252=EDGE_CURVE('',#41486,#41487,#22436,.T.);
#53253=EDGE_CURVE('',#41488,#41487,#33677,.T.);
#53254=EDGE_CURVE('',#41489,#41488,#33678,.T.);
#53255=EDGE_CURVE('',#41490,#41489,#33679,.T.);
#53256=EDGE_CURVE('',#41490,#41485,#22437,.T.);
#53257=EDGE_CURVE('',#41488,#41491,#22438,.T.);
#53258=EDGE_CURVE('',#41491,#41492,#33680,.T.);
#53259=EDGE_CURVE('',#41492,#41489,#22439,.T.);
#53260=EDGE_CURVE('',#41083,#41474,#33681,.T.);
#53261=EDGE_CURVE('',#41473,#41084,#33682,.T.);
#53262=EDGE_CURVE('',#41491,#40723,#1508,.T.);
#53263=EDGE_CURVE('',#40722,#41492,#1509,.T.);
#53264=EDGE_CURVE('',#41483,#41486,#1510,.T.);
#53265=EDGE_CURVE('',#41485,#41484,#1511,.T.);
#53266=EDGE_CURVE('',#41479,#41482,#1512,.T.);
#53267=EDGE_CURVE('',#41481,#41480,#1513,.T.);
#53268=EDGE_CURVE('',#41493,#41494,#33683,.T.);
#53269=EDGE_CURVE('',#41494,#41495,#22440,.T.);
#53270=EDGE_CURVE('',#41496,#41495,#33684,.T.);
#53271=EDGE_CURVE('',#41497,#41496,#33685,.T.);
#53272=EDGE_CURVE('',#41498,#41497,#33686,.T.);
#53273=EDGE_CURVE('',#41498,#41493,#22441,.T.);
#53274=EDGE_CURVE('',#41496,#41499,#22442,.T.);
#53275=EDGE_CURVE('',#41499,#41500,#33687,.T.);
#53276=EDGE_CURVE('',#41500,#41497,#22443,.T.);
#53277=EDGE_CURVE('',#41501,#41502,#33688,.T.);
#53278=EDGE_CURVE('',#41502,#41503,#22444,.T.);
#53279=EDGE_CURVE('',#41503,#41504,#33689,.T.);
#53280=EDGE_CURVE('',#41504,#41501,#22445,.T.);
#53281=EDGE_CURVE('',#41505,#41506,#33690,.T.);
#53282=EDGE_CURVE('',#41506,#41507,#22446,.T.);
#53283=EDGE_CURVE('',#41508,#41507,#33691,.T.);
#53284=EDGE_CURVE('',#41509,#41508,#33692,.T.);
#53285=EDGE_CURVE('',#41510,#41509,#33693,.T.);
#53286=EDGE_CURVE('',#41510,#41505,#22447,.T.);
#53287=EDGE_CURVE('',#41508,#41511,#22448,.T.);
#53288=EDGE_CURVE('',#41511,#41512,#33694,.T.);
#53289=EDGE_CURVE('',#41512,#41509,#22449,.T.);
#53290=EDGE_CURVE('',#41089,#41494,#33695,.T.);
#53291=EDGE_CURVE('',#41493,#41090,#33696,.T.);
#53292=EDGE_CURVE('',#41511,#40717,#1514,.T.);
#53293=EDGE_CURVE('',#40716,#41512,#1515,.T.);
#53294=EDGE_CURVE('',#41503,#41506,#1516,.T.);
#53295=EDGE_CURVE('',#41505,#41504,#1517,.T.);
#53296=EDGE_CURVE('',#41499,#41502,#1518,.T.);
#53297=EDGE_CURVE('',#41501,#41500,#1519,.T.);
#53298=EDGE_CURVE('',#41513,#41514,#33697,.T.);
#53299=EDGE_CURVE('',#41514,#41515,#22450,.T.);
#53300=EDGE_CURVE('',#41516,#41515,#33698,.T.);
#53301=EDGE_CURVE('',#41517,#41516,#33699,.T.);
#53302=EDGE_CURVE('',#41518,#41517,#33700,.T.);
#53303=EDGE_CURVE('',#41518,#41513,#22451,.T.);
#53304=EDGE_CURVE('',#41516,#41519,#22452,.T.);
#53305=EDGE_CURVE('',#41519,#41520,#33701,.T.);
#53306=EDGE_CURVE('',#41520,#41517,#22453,.T.);
#53307=EDGE_CURVE('',#41521,#41522,#33702,.T.);
#53308=EDGE_CURVE('',#41522,#41523,#22454,.T.);
#53309=EDGE_CURVE('',#41523,#41524,#33703,.T.);
#53310=EDGE_CURVE('',#41524,#41521,#22455,.T.);
#53311=EDGE_CURVE('',#41525,#41526,#33704,.T.);
#53312=EDGE_CURVE('',#41526,#41527,#22456,.T.);
#53313=EDGE_CURVE('',#41528,#41527,#33705,.T.);
#53314=EDGE_CURVE('',#41529,#41528,#33706,.T.);
#53315=EDGE_CURVE('',#41530,#41529,#33707,.T.);
#53316=EDGE_CURVE('',#41530,#41525,#22457,.T.);
#53317=EDGE_CURVE('',#41528,#41531,#22458,.T.);
#53318=EDGE_CURVE('',#41531,#41532,#33708,.T.);
#53319=EDGE_CURVE('',#41532,#41529,#22459,.T.);
#53320=EDGE_CURVE('',#41095,#41514,#33709,.T.);
#53321=EDGE_CURVE('',#41513,#41096,#33710,.T.);
#53322=EDGE_CURVE('',#41531,#40711,#1520,.T.);
#53323=EDGE_CURVE('',#40710,#41532,#1521,.T.);
#53324=EDGE_CURVE('',#41523,#41526,#1522,.T.);
#53325=EDGE_CURVE('',#41525,#41524,#1523,.T.);
#53326=EDGE_CURVE('',#41519,#41522,#1524,.T.);
#53327=EDGE_CURVE('',#41521,#41520,#1525,.T.);
#53328=EDGE_CURVE('',#41533,#41534,#33711,.T.);
#53329=EDGE_CURVE('',#41534,#41535,#22460,.T.);
#53330=EDGE_CURVE('',#41536,#41535,#33712,.T.);
#53331=EDGE_CURVE('',#41537,#41536,#33713,.T.);
#53332=EDGE_CURVE('',#41538,#41537,#33714,.T.);
#53333=EDGE_CURVE('',#41538,#41533,#22461,.T.);
#53334=EDGE_CURVE('',#41536,#41539,#22462,.T.);
#53335=EDGE_CURVE('',#41539,#41540,#33715,.T.);
#53336=EDGE_CURVE('',#41540,#41537,#22463,.T.);
#53337=EDGE_CURVE('',#41541,#41542,#33716,.T.);
#53338=EDGE_CURVE('',#41542,#41543,#22464,.T.);
#53339=EDGE_CURVE('',#41543,#41544,#33717,.T.);
#53340=EDGE_CURVE('',#41544,#41541,#22465,.T.);
#53341=EDGE_CURVE('',#41545,#41546,#33718,.T.);
#53342=EDGE_CURVE('',#41546,#41547,#22466,.T.);
#53343=EDGE_CURVE('',#41548,#41547,#33719,.T.);
#53344=EDGE_CURVE('',#41549,#41548,#33720,.T.);
#53345=EDGE_CURVE('',#41550,#41549,#33721,.T.);
#53346=EDGE_CURVE('',#41550,#41545,#22467,.T.);
#53347=EDGE_CURVE('',#41548,#41551,#22468,.T.);
#53348=EDGE_CURVE('',#41551,#41552,#33722,.T.);
#53349=EDGE_CURVE('',#41552,#41549,#22469,.T.);
#53350=EDGE_CURVE('',#41101,#41534,#33723,.T.);
#53351=EDGE_CURVE('',#41533,#41102,#33724,.T.);
#53352=EDGE_CURVE('',#41551,#40705,#1526,.T.);
#53353=EDGE_CURVE('',#40704,#41552,#1527,.T.);
#53354=EDGE_CURVE('',#41543,#41546,#1528,.T.);
#53355=EDGE_CURVE('',#41545,#41544,#1529,.T.);
#53356=EDGE_CURVE('',#41539,#41542,#1530,.T.);
#53357=EDGE_CURVE('',#41541,#41540,#1531,.T.);
#53358=EDGE_CURVE('',#41553,#41554,#33725,.T.);
#53359=EDGE_CURVE('',#41554,#41555,#22470,.T.);
#53360=EDGE_CURVE('',#41556,#41555,#33726,.T.);
#53361=EDGE_CURVE('',#41557,#41556,#33727,.T.);
#53362=EDGE_CURVE('',#41558,#41557,#33728,.T.);
#53363=EDGE_CURVE('',#41558,#41553,#22471,.T.);
#53364=EDGE_CURVE('',#41556,#41559,#22472,.T.);
#53365=EDGE_CURVE('',#41559,#41560,#33729,.T.);
#53366=EDGE_CURVE('',#41560,#41557,#22473,.T.);
#53367=EDGE_CURVE('',#41561,#41562,#33730,.T.);
#53368=EDGE_CURVE('',#41562,#41563,#22474,.T.);
#53369=EDGE_CURVE('',#41563,#41564,#33731,.T.);
#53370=EDGE_CURVE('',#41564,#41561,#22475,.T.);
#53371=EDGE_CURVE('',#41565,#41566,#33732,.T.);
#53372=EDGE_CURVE('',#41566,#41567,#22476,.T.);
#53373=EDGE_CURVE('',#41568,#41567,#33733,.T.);
#53374=EDGE_CURVE('',#41569,#41568,#33734,.T.);
#53375=EDGE_CURVE('',#41570,#41569,#33735,.T.);
#53376=EDGE_CURVE('',#41570,#41565,#22477,.T.);
#53377=EDGE_CURVE('',#41568,#41571,#22478,.T.);
#53378=EDGE_CURVE('',#41571,#41572,#33736,.T.);
#53379=EDGE_CURVE('',#41572,#41569,#22479,.T.);
#53380=EDGE_CURVE('',#41107,#41554,#33737,.T.);
#53381=EDGE_CURVE('',#41553,#41108,#33738,.T.);
#53382=EDGE_CURVE('',#41571,#40699,#1532,.T.);
#53383=EDGE_CURVE('',#40698,#41572,#1533,.T.);
#53384=EDGE_CURVE('',#41563,#41566,#1534,.T.);
#53385=EDGE_CURVE('',#41565,#41564,#1535,.T.);
#53386=EDGE_CURVE('',#41559,#41562,#1536,.T.);
#53387=EDGE_CURVE('',#41561,#41560,#1537,.T.);
#53388=EDGE_CURVE('',#41573,#41574,#33739,.T.);
#53389=EDGE_CURVE('',#41574,#41575,#22480,.T.);
#53390=EDGE_CURVE('',#41576,#41575,#33740,.T.);
#53391=EDGE_CURVE('',#41577,#41576,#33741,.T.);
#53392=EDGE_CURVE('',#41578,#41577,#33742,.T.);
#53393=EDGE_CURVE('',#41578,#41573,#22481,.T.);
#53394=EDGE_CURVE('',#41576,#41579,#22482,.T.);
#53395=EDGE_CURVE('',#41579,#41580,#33743,.T.);
#53396=EDGE_CURVE('',#41580,#41577,#22483,.T.);
#53397=EDGE_CURVE('',#41581,#41582,#33744,.T.);
#53398=EDGE_CURVE('',#41582,#41583,#22484,.T.);
#53399=EDGE_CURVE('',#41583,#41584,#33745,.T.);
#53400=EDGE_CURVE('',#41584,#41581,#22485,.T.);
#53401=EDGE_CURVE('',#41585,#41586,#33746,.T.);
#53402=EDGE_CURVE('',#41586,#41587,#22486,.T.);
#53403=EDGE_CURVE('',#41588,#41587,#33747,.T.);
#53404=EDGE_CURVE('',#41589,#41588,#33748,.T.);
#53405=EDGE_CURVE('',#41590,#41589,#33749,.T.);
#53406=EDGE_CURVE('',#41590,#41585,#22487,.T.);
#53407=EDGE_CURVE('',#41588,#41591,#22488,.T.);
#53408=EDGE_CURVE('',#41591,#41592,#33750,.T.);
#53409=EDGE_CURVE('',#41592,#41589,#22489,.T.);
#53410=EDGE_CURVE('',#41113,#41574,#33751,.T.);
#53411=EDGE_CURVE('',#41573,#41114,#33752,.T.);
#53412=EDGE_CURVE('',#41591,#40693,#1538,.T.);
#53413=EDGE_CURVE('',#40692,#41592,#1539,.T.);
#53414=EDGE_CURVE('',#41583,#41586,#1540,.T.);
#53415=EDGE_CURVE('',#41585,#41584,#1541,.T.);
#53416=EDGE_CURVE('',#41579,#41582,#1542,.T.);
#53417=EDGE_CURVE('',#41581,#41580,#1543,.T.);
#53418=EDGE_CURVE('',#41593,#41594,#33753,.T.);
#53419=EDGE_CURVE('',#41594,#41595,#22490,.T.);
#53420=EDGE_CURVE('',#41596,#41595,#33754,.T.);
#53421=EDGE_CURVE('',#41597,#41596,#33755,.T.);
#53422=EDGE_CURVE('',#41598,#41597,#33756,.T.);
#53423=EDGE_CURVE('',#41598,#41593,#22491,.T.);
#53424=EDGE_CURVE('',#41596,#41599,#22492,.T.);
#53425=EDGE_CURVE('',#41599,#41600,#33757,.T.);
#53426=EDGE_CURVE('',#41600,#41597,#22493,.T.);
#53427=EDGE_CURVE('',#41601,#41602,#33758,.T.);
#53428=EDGE_CURVE('',#41602,#41603,#22494,.T.);
#53429=EDGE_CURVE('',#41603,#41604,#33759,.T.);
#53430=EDGE_CURVE('',#41604,#41601,#22495,.T.);
#53431=EDGE_CURVE('',#41605,#41606,#33760,.T.);
#53432=EDGE_CURVE('',#41606,#41607,#22496,.T.);
#53433=EDGE_CURVE('',#41608,#41607,#33761,.T.);
#53434=EDGE_CURVE('',#41609,#41608,#33762,.T.);
#53435=EDGE_CURVE('',#41610,#41609,#33763,.T.);
#53436=EDGE_CURVE('',#41610,#41605,#22497,.T.);
#53437=EDGE_CURVE('',#41608,#41611,#22498,.T.);
#53438=EDGE_CURVE('',#41611,#41612,#33764,.T.);
#53439=EDGE_CURVE('',#41612,#41609,#22499,.T.);
#53440=EDGE_CURVE('',#41119,#41594,#33765,.T.);
#53441=EDGE_CURVE('',#41593,#41120,#33766,.T.);
#53442=EDGE_CURVE('',#41611,#40687,#1544,.T.);
#53443=EDGE_CURVE('',#40686,#41612,#1545,.T.);
#53444=EDGE_CURVE('',#41603,#41606,#1546,.T.);
#53445=EDGE_CURVE('',#41605,#41604,#1547,.T.);
#53446=EDGE_CURVE('',#41599,#41602,#1548,.T.);
#53447=EDGE_CURVE('',#41601,#41600,#1549,.T.);
#53448=EDGE_CURVE('',#41613,#41614,#33767,.T.);
#53449=EDGE_CURVE('',#41614,#41615,#22500,.T.);
#53450=EDGE_CURVE('',#41616,#41615,#33768,.T.);
#53451=EDGE_CURVE('',#41617,#41616,#33769,.T.);
#53452=EDGE_CURVE('',#41618,#41617,#33770,.T.);
#53453=EDGE_CURVE('',#41618,#41613,#22501,.T.);
#53454=EDGE_CURVE('',#41616,#41619,#22502,.T.);
#53455=EDGE_CURVE('',#41619,#41620,#33771,.T.);
#53456=EDGE_CURVE('',#41620,#41617,#22503,.T.);
#53457=EDGE_CURVE('',#41621,#41622,#33772,.T.);
#53458=EDGE_CURVE('',#41622,#41623,#22504,.T.);
#53459=EDGE_CURVE('',#41623,#41624,#33773,.T.);
#53460=EDGE_CURVE('',#41624,#41621,#22505,.T.);
#53461=EDGE_CURVE('',#41625,#41626,#33774,.T.);
#53462=EDGE_CURVE('',#41626,#41627,#22506,.T.);
#53463=EDGE_CURVE('',#41628,#41627,#33775,.T.);
#53464=EDGE_CURVE('',#41629,#41628,#33776,.T.);
#53465=EDGE_CURVE('',#41630,#41629,#33777,.T.);
#53466=EDGE_CURVE('',#41630,#41625,#22507,.T.);
#53467=EDGE_CURVE('',#41628,#41631,#22508,.T.);
#53468=EDGE_CURVE('',#41631,#41632,#33778,.T.);
#53469=EDGE_CURVE('',#41632,#41629,#22509,.T.);
#53470=EDGE_CURVE('',#41125,#41614,#33779,.T.);
#53471=EDGE_CURVE('',#41613,#41126,#33780,.T.);
#53472=EDGE_CURVE('',#41631,#40681,#1550,.T.);
#53473=EDGE_CURVE('',#40680,#41632,#1551,.T.);
#53474=EDGE_CURVE('',#41623,#41626,#1552,.T.);
#53475=EDGE_CURVE('',#41625,#41624,#1553,.T.);
#53476=EDGE_CURVE('',#41619,#41622,#1554,.T.);
#53477=EDGE_CURVE('',#41621,#41620,#1555,.T.);
#53478=EDGE_CURVE('',#41633,#41634,#33781,.T.);
#53479=EDGE_CURVE('',#41634,#41635,#22510,.T.);
#53480=EDGE_CURVE('',#41636,#41635,#33782,.T.);
#53481=EDGE_CURVE('',#41637,#41636,#33783,.T.);
#53482=EDGE_CURVE('',#41638,#41637,#33784,.T.);
#53483=EDGE_CURVE('',#41638,#41633,#22511,.T.);
#53484=EDGE_CURVE('',#41636,#41639,#22512,.T.);
#53485=EDGE_CURVE('',#41639,#41640,#33785,.T.);
#53486=EDGE_CURVE('',#41640,#41637,#22513,.T.);
#53487=EDGE_CURVE('',#41641,#41642,#33786,.T.);
#53488=EDGE_CURVE('',#41642,#41643,#22514,.T.);
#53489=EDGE_CURVE('',#41643,#41644,#33787,.T.);
#53490=EDGE_CURVE('',#41644,#41641,#22515,.T.);
#53491=EDGE_CURVE('',#41645,#41646,#33788,.T.);
#53492=EDGE_CURVE('',#41646,#41647,#22516,.T.);
#53493=EDGE_CURVE('',#41648,#41647,#33789,.T.);
#53494=EDGE_CURVE('',#41649,#41648,#33790,.T.);
#53495=EDGE_CURVE('',#41650,#41649,#33791,.T.);
#53496=EDGE_CURVE('',#41650,#41645,#22517,.T.);
#53497=EDGE_CURVE('',#41648,#41651,#22518,.T.);
#53498=EDGE_CURVE('',#41651,#41652,#33792,.T.);
#53499=EDGE_CURVE('',#41652,#41649,#22519,.T.);
#53500=EDGE_CURVE('',#41131,#41634,#33793,.T.);
#53501=EDGE_CURVE('',#41633,#41132,#33794,.T.);
#53502=EDGE_CURVE('',#41651,#40675,#1556,.T.);
#53503=EDGE_CURVE('',#40674,#41652,#1557,.T.);
#53504=EDGE_CURVE('',#41643,#41646,#1558,.T.);
#53505=EDGE_CURVE('',#41645,#41644,#1559,.T.);
#53506=EDGE_CURVE('',#41639,#41642,#1560,.T.);
#53507=EDGE_CURVE('',#41641,#41640,#1561,.T.);
#53508=EDGE_CURVE('',#41653,#41654,#33795,.T.);
#53509=EDGE_CURVE('',#41654,#41655,#22520,.T.);
#53510=EDGE_CURVE('',#41656,#41655,#33796,.T.);
#53511=EDGE_CURVE('',#41657,#41656,#33797,.T.);
#53512=EDGE_CURVE('',#41658,#41657,#33798,.T.);
#53513=EDGE_CURVE('',#41658,#41653,#22521,.T.);
#53514=EDGE_CURVE('',#41656,#41659,#22522,.T.);
#53515=EDGE_CURVE('',#41659,#41660,#33799,.T.);
#53516=EDGE_CURVE('',#41660,#41657,#22523,.T.);
#53517=EDGE_CURVE('',#41661,#41662,#33800,.T.);
#53518=EDGE_CURVE('',#41662,#41663,#22524,.T.);
#53519=EDGE_CURVE('',#41663,#41664,#33801,.T.);
#53520=EDGE_CURVE('',#41664,#41661,#22525,.T.);
#53521=EDGE_CURVE('',#41665,#41666,#33802,.T.);
#53522=EDGE_CURVE('',#41666,#41667,#22526,.T.);
#53523=EDGE_CURVE('',#41668,#41667,#33803,.T.);
#53524=EDGE_CURVE('',#41669,#41668,#33804,.T.);
#53525=EDGE_CURVE('',#41670,#41669,#33805,.T.);
#53526=EDGE_CURVE('',#41670,#41665,#22527,.T.);
#53527=EDGE_CURVE('',#41668,#41671,#22528,.T.);
#53528=EDGE_CURVE('',#41671,#41672,#33806,.T.);
#53529=EDGE_CURVE('',#41672,#41669,#22529,.T.);
#53530=EDGE_CURVE('',#41137,#41654,#33807,.T.);
#53531=EDGE_CURVE('',#41653,#41138,#33808,.T.);
#53532=EDGE_CURVE('',#41671,#40669,#1562,.T.);
#53533=EDGE_CURVE('',#40668,#41672,#1563,.T.);
#53534=EDGE_CURVE('',#41663,#41666,#1564,.T.);
#53535=EDGE_CURVE('',#41665,#41664,#1565,.T.);
#53536=EDGE_CURVE('',#41659,#41662,#1566,.T.);
#53537=EDGE_CURVE('',#41661,#41660,#1567,.T.);
#53538=EDGE_CURVE('',#41673,#41674,#33809,.T.);
#53539=EDGE_CURVE('',#41674,#41675,#22530,.T.);
#53540=EDGE_CURVE('',#41676,#41675,#33810,.T.);
#53541=EDGE_CURVE('',#41677,#41676,#33811,.T.);
#53542=EDGE_CURVE('',#41678,#41677,#33812,.T.);
#53543=EDGE_CURVE('',#41678,#41673,#22531,.T.);
#53544=EDGE_CURVE('',#41676,#41679,#22532,.T.);
#53545=EDGE_CURVE('',#41679,#41680,#33813,.T.);
#53546=EDGE_CURVE('',#41680,#41677,#22533,.T.);
#53547=EDGE_CURVE('',#41681,#41682,#33814,.T.);
#53548=EDGE_CURVE('',#41682,#41683,#22534,.T.);
#53549=EDGE_CURVE('',#41683,#41684,#33815,.T.);
#53550=EDGE_CURVE('',#41684,#41681,#22535,.T.);
#53551=EDGE_CURVE('',#41685,#41686,#33816,.T.);
#53552=EDGE_CURVE('',#41686,#41687,#22536,.T.);
#53553=EDGE_CURVE('',#41688,#41687,#33817,.T.);
#53554=EDGE_CURVE('',#41689,#41688,#33818,.T.);
#53555=EDGE_CURVE('',#41690,#41689,#33819,.T.);
#53556=EDGE_CURVE('',#41690,#41685,#22537,.T.);
#53557=EDGE_CURVE('',#41688,#41691,#22538,.T.);
#53558=EDGE_CURVE('',#41691,#41692,#33820,.T.);
#53559=EDGE_CURVE('',#41692,#41689,#22539,.T.);
#53560=EDGE_CURVE('',#41143,#41674,#33821,.T.);
#53561=EDGE_CURVE('',#41673,#41144,#33822,.T.);
#53562=EDGE_CURVE('',#41691,#40663,#1568,.T.);
#53563=EDGE_CURVE('',#40662,#41692,#1569,.T.);
#53564=EDGE_CURVE('',#41683,#41686,#1570,.T.);
#53565=EDGE_CURVE('',#41685,#41684,#1571,.T.);
#53566=EDGE_CURVE('',#41679,#41682,#1572,.T.);
#53567=EDGE_CURVE('',#41681,#41680,#1573,.T.);
#53568=EDGE_CURVE('',#41693,#41694,#33823,.T.);
#53569=EDGE_CURVE('',#41694,#41695,#22540,.T.);
#53570=EDGE_CURVE('',#41696,#41695,#33824,.T.);
#53571=EDGE_CURVE('',#41697,#41696,#33825,.T.);
#53572=EDGE_CURVE('',#41698,#41697,#33826,.T.);
#53573=EDGE_CURVE('',#41698,#41693,#22541,.T.);
#53574=EDGE_CURVE('',#41696,#41699,#22542,.T.);
#53575=EDGE_CURVE('',#41699,#41700,#33827,.T.);
#53576=EDGE_CURVE('',#41700,#41697,#22543,.T.);
#53577=EDGE_CURVE('',#41701,#41702,#33828,.T.);
#53578=EDGE_CURVE('',#41702,#41703,#22544,.T.);
#53579=EDGE_CURVE('',#41703,#41704,#33829,.T.);
#53580=EDGE_CURVE('',#41704,#41701,#22545,.T.);
#53581=EDGE_CURVE('',#41705,#41706,#33830,.T.);
#53582=EDGE_CURVE('',#41706,#41707,#22546,.T.);
#53583=EDGE_CURVE('',#41708,#41707,#33831,.T.);
#53584=EDGE_CURVE('',#41709,#41708,#33832,.T.);
#53585=EDGE_CURVE('',#41710,#41709,#33833,.T.);
#53586=EDGE_CURVE('',#41710,#41705,#22547,.T.);
#53587=EDGE_CURVE('',#41708,#41711,#22548,.T.);
#53588=EDGE_CURVE('',#41711,#41712,#33834,.T.);
#53589=EDGE_CURVE('',#41712,#41709,#22549,.T.);
#53590=EDGE_CURVE('',#41149,#41694,#33835,.T.);
#53591=EDGE_CURVE('',#41693,#41150,#33836,.T.);
#53592=EDGE_CURVE('',#41711,#40657,#1574,.T.);
#53593=EDGE_CURVE('',#40656,#41712,#1575,.T.);
#53594=EDGE_CURVE('',#41703,#41706,#1576,.T.);
#53595=EDGE_CURVE('',#41705,#41704,#1577,.T.);
#53596=EDGE_CURVE('',#41699,#41702,#1578,.T.);
#53597=EDGE_CURVE('',#41701,#41700,#1579,.T.);
#53598=EDGE_CURVE('',#41713,#41714,#33837,.T.);
#53599=EDGE_CURVE('',#41714,#41715,#22550,.T.);
#53600=EDGE_CURVE('',#41716,#41715,#33838,.T.);
#53601=EDGE_CURVE('',#41717,#41716,#33839,.T.);
#53602=EDGE_CURVE('',#41718,#41717,#33840,.T.);
#53603=EDGE_CURVE('',#41718,#41713,#22551,.T.);
#53604=EDGE_CURVE('',#41716,#41719,#22552,.T.);
#53605=EDGE_CURVE('',#41719,#41720,#33841,.T.);
#53606=EDGE_CURVE('',#41720,#41717,#22553,.T.);
#53607=EDGE_CURVE('',#41721,#41722,#33842,.T.);
#53608=EDGE_CURVE('',#41722,#41723,#22554,.T.);
#53609=EDGE_CURVE('',#41723,#41724,#33843,.T.);
#53610=EDGE_CURVE('',#41724,#41721,#22555,.T.);
#53611=EDGE_CURVE('',#41725,#41726,#33844,.T.);
#53612=EDGE_CURVE('',#41726,#41727,#22556,.T.);
#53613=EDGE_CURVE('',#41728,#41727,#33845,.T.);
#53614=EDGE_CURVE('',#41729,#41728,#33846,.T.);
#53615=EDGE_CURVE('',#41730,#41729,#33847,.T.);
#53616=EDGE_CURVE('',#41730,#41725,#22557,.T.);
#53617=EDGE_CURVE('',#41728,#41731,#22558,.T.);
#53618=EDGE_CURVE('',#41731,#41732,#33848,.T.);
#53619=EDGE_CURVE('',#41732,#41729,#22559,.T.);
#53620=EDGE_CURVE('',#41155,#41714,#33849,.T.);
#53621=EDGE_CURVE('',#41713,#41156,#33850,.T.);
#53622=EDGE_CURVE('',#41731,#40651,#1580,.T.);
#53623=EDGE_CURVE('',#40650,#41732,#1581,.T.);
#53624=EDGE_CURVE('',#41723,#41726,#1582,.T.);
#53625=EDGE_CURVE('',#41725,#41724,#1583,.T.);
#53626=EDGE_CURVE('',#41719,#41722,#1584,.T.);
#53627=EDGE_CURVE('',#41721,#41720,#1585,.T.);
#53628=EDGE_CURVE('',#41733,#41734,#33851,.T.);
#53629=EDGE_CURVE('',#41734,#41735,#22560,.T.);
#53630=EDGE_CURVE('',#41736,#41735,#33852,.T.);
#53631=EDGE_CURVE('',#41737,#41736,#33853,.T.);
#53632=EDGE_CURVE('',#41738,#41737,#33854,.T.);
#53633=EDGE_CURVE('',#41738,#41733,#22561,.T.);
#53634=EDGE_CURVE('',#41736,#41739,#22562,.T.);
#53635=EDGE_CURVE('',#41739,#41740,#33855,.T.);
#53636=EDGE_CURVE('',#41740,#41737,#22563,.T.);
#53637=EDGE_CURVE('',#41741,#41742,#33856,.T.);
#53638=EDGE_CURVE('',#41742,#41743,#22564,.T.);
#53639=EDGE_CURVE('',#41743,#41744,#33857,.T.);
#53640=EDGE_CURVE('',#41744,#41741,#22565,.T.);
#53641=EDGE_CURVE('',#41745,#41746,#33858,.T.);
#53642=EDGE_CURVE('',#41746,#41747,#22566,.T.);
#53643=EDGE_CURVE('',#41748,#41747,#33859,.T.);
#53644=EDGE_CURVE('',#41749,#41748,#33860,.T.);
#53645=EDGE_CURVE('',#41750,#41749,#33861,.T.);
#53646=EDGE_CURVE('',#41750,#41745,#22567,.T.);
#53647=EDGE_CURVE('',#41748,#41751,#22568,.T.);
#53648=EDGE_CURVE('',#41751,#41752,#33862,.T.);
#53649=EDGE_CURVE('',#41752,#41749,#22569,.T.);
#53650=EDGE_CURVE('',#41161,#41734,#33863,.T.);
#53651=EDGE_CURVE('',#41733,#41162,#33864,.T.);
#53652=EDGE_CURVE('',#41751,#40645,#1586,.T.);
#53653=EDGE_CURVE('',#40644,#41752,#1587,.T.);
#53654=EDGE_CURVE('',#41743,#41746,#1588,.T.);
#53655=EDGE_CURVE('',#41745,#41744,#1589,.T.);
#53656=EDGE_CURVE('',#41739,#41742,#1590,.T.);
#53657=EDGE_CURVE('',#41741,#41740,#1591,.T.);
#53658=EDGE_CURVE('',#41753,#41754,#33865,.T.);
#53659=EDGE_CURVE('',#41754,#41755,#22570,.T.);
#53660=EDGE_CURVE('',#41756,#41755,#33866,.T.);
#53661=EDGE_CURVE('',#41757,#41756,#33867,.T.);
#53662=EDGE_CURVE('',#41758,#41757,#33868,.T.);
#53663=EDGE_CURVE('',#41758,#41753,#22571,.T.);
#53664=EDGE_CURVE('',#41756,#41759,#22572,.T.);
#53665=EDGE_CURVE('',#41759,#41760,#33869,.T.);
#53666=EDGE_CURVE('',#41760,#41757,#22573,.T.);
#53667=EDGE_CURVE('',#41761,#41762,#33870,.T.);
#53668=EDGE_CURVE('',#41762,#41763,#22574,.T.);
#53669=EDGE_CURVE('',#41763,#41764,#33871,.T.);
#53670=EDGE_CURVE('',#41764,#41761,#22575,.T.);
#53671=EDGE_CURVE('',#41765,#41766,#33872,.T.);
#53672=EDGE_CURVE('',#41766,#41767,#22576,.T.);
#53673=EDGE_CURVE('',#41768,#41767,#33873,.T.);
#53674=EDGE_CURVE('',#41769,#41768,#33874,.T.);
#53675=EDGE_CURVE('',#41770,#41769,#33875,.T.);
#53676=EDGE_CURVE('',#41770,#41765,#22577,.T.);
#53677=EDGE_CURVE('',#41768,#41771,#22578,.T.);
#53678=EDGE_CURVE('',#41771,#41772,#33876,.T.);
#53679=EDGE_CURVE('',#41772,#41769,#22579,.T.);
#53680=EDGE_CURVE('',#41167,#41754,#33877,.T.);
#53681=EDGE_CURVE('',#41753,#41168,#33878,.T.);
#53682=EDGE_CURVE('',#41771,#40639,#1592,.T.);
#53683=EDGE_CURVE('',#40638,#41772,#1593,.T.);
#53684=EDGE_CURVE('',#41763,#41766,#1594,.T.);
#53685=EDGE_CURVE('',#41765,#41764,#1595,.T.);
#53686=EDGE_CURVE('',#41759,#41762,#1596,.T.);
#53687=EDGE_CURVE('',#41761,#41760,#1597,.T.);
#53688=EDGE_CURVE('',#41773,#41774,#33879,.T.);
#53689=EDGE_CURVE('',#41774,#41775,#22580,.T.);
#53690=EDGE_CURVE('',#41776,#41775,#33880,.T.);
#53691=EDGE_CURVE('',#41777,#41776,#33881,.T.);
#53692=EDGE_CURVE('',#41778,#41777,#33882,.T.);
#53693=EDGE_CURVE('',#41778,#41773,#22581,.T.);
#53694=EDGE_CURVE('',#41776,#41779,#22582,.T.);
#53695=EDGE_CURVE('',#41779,#41780,#33883,.T.);
#53696=EDGE_CURVE('',#41780,#41777,#22583,.T.);
#53697=EDGE_CURVE('',#41781,#41782,#33884,.T.);
#53698=EDGE_CURVE('',#41782,#41783,#22584,.T.);
#53699=EDGE_CURVE('',#41783,#41784,#33885,.T.);
#53700=EDGE_CURVE('',#41784,#41781,#22585,.T.);
#53701=EDGE_CURVE('',#41785,#41786,#33886,.T.);
#53702=EDGE_CURVE('',#41786,#41787,#22586,.T.);
#53703=EDGE_CURVE('',#41788,#41787,#33887,.T.);
#53704=EDGE_CURVE('',#41789,#41788,#33888,.T.);
#53705=EDGE_CURVE('',#41790,#41789,#33889,.T.);
#53706=EDGE_CURVE('',#41790,#41785,#22587,.T.);
#53707=EDGE_CURVE('',#41788,#41791,#22588,.T.);
#53708=EDGE_CURVE('',#41791,#41792,#33890,.T.);
#53709=EDGE_CURVE('',#41792,#41789,#22589,.T.);
#53710=EDGE_CURVE('',#40814,#41774,#33891,.T.);
#53711=EDGE_CURVE('',#41773,#40815,#33892,.T.);
#53712=EDGE_CURVE('',#41791,#40635,#1598,.T.);
#53713=EDGE_CURVE('',#40634,#41792,#1599,.T.);
#53714=EDGE_CURVE('',#41783,#41786,#1600,.T.);
#53715=EDGE_CURVE('',#41785,#41784,#1601,.T.);
#53716=EDGE_CURVE('',#41779,#41782,#1602,.T.);
#53717=EDGE_CURVE('',#41781,#41780,#1603,.T.);
#53718=EDGE_CURVE('',#41793,#41794,#33893,.T.);
#53719=EDGE_CURVE('',#41794,#41795,#22590,.T.);
#53720=EDGE_CURVE('',#41796,#41795,#33894,.T.);
#53721=EDGE_CURVE('',#41797,#41796,#33895,.T.);
#53722=EDGE_CURVE('',#41798,#41797,#33896,.T.);
#53723=EDGE_CURVE('',#41798,#41793,#22591,.T.);
#53724=EDGE_CURVE('',#41796,#41799,#22592,.T.);
#53725=EDGE_CURVE('',#41799,#41800,#33897,.T.);
#53726=EDGE_CURVE('',#41800,#41797,#22593,.T.);
#53727=EDGE_CURVE('',#41801,#41802,#33898,.T.);
#53728=EDGE_CURVE('',#41802,#41803,#22594,.T.);
#53729=EDGE_CURVE('',#41803,#41804,#33899,.T.);
#53730=EDGE_CURVE('',#41804,#41801,#22595,.T.);
#53731=EDGE_CURVE('',#41805,#41806,#33900,.T.);
#53732=EDGE_CURVE('',#41806,#41807,#22596,.T.);
#53733=EDGE_CURVE('',#41808,#41807,#33901,.T.);
#53734=EDGE_CURVE('',#41809,#41808,#33902,.T.);
#53735=EDGE_CURVE('',#41810,#41809,#33903,.T.);
#53736=EDGE_CURVE('',#41810,#41805,#22597,.T.);
#53737=EDGE_CURVE('',#41808,#41811,#22598,.T.);
#53738=EDGE_CURVE('',#41811,#41812,#33904,.T.);
#53739=EDGE_CURVE('',#41812,#41809,#22599,.T.);
#53740=EDGE_CURVE('',#40820,#41794,#33905,.T.);
#53741=EDGE_CURVE('',#41793,#40821,#33906,.T.);
#53742=EDGE_CURVE('',#41811,#40629,#1604,.T.);
#53743=EDGE_CURVE('',#40628,#41812,#1605,.T.);
#53744=EDGE_CURVE('',#41803,#41806,#1606,.T.);
#53745=EDGE_CURVE('',#41805,#41804,#1607,.T.);
#53746=EDGE_CURVE('',#41799,#41802,#1608,.T.);
#53747=EDGE_CURVE('',#41801,#41800,#1609,.T.);
#53748=EDGE_CURVE('',#41813,#41814,#33907,.T.);
#53749=EDGE_CURVE('',#41814,#41815,#22600,.T.);
#53750=EDGE_CURVE('',#41816,#41815,#33908,.T.);
#53751=EDGE_CURVE('',#41817,#41816,#33909,.T.);
#53752=EDGE_CURVE('',#41818,#41817,#33910,.T.);
#53753=EDGE_CURVE('',#41818,#41813,#22601,.T.);
#53754=EDGE_CURVE('',#41816,#41819,#22602,.T.);
#53755=EDGE_CURVE('',#41819,#41820,#33911,.T.);
#53756=EDGE_CURVE('',#41820,#41817,#22603,.T.);
#53757=EDGE_CURVE('',#41821,#41822,#33912,.T.);
#53758=EDGE_CURVE('',#41822,#41823,#22604,.T.);
#53759=EDGE_CURVE('',#41823,#41824,#33913,.T.);
#53760=EDGE_CURVE('',#41824,#41821,#22605,.T.);
#53761=EDGE_CURVE('',#41825,#41826,#33914,.T.);
#53762=EDGE_CURVE('',#41826,#41827,#22606,.T.);
#53763=EDGE_CURVE('',#41828,#41827,#33915,.T.);
#53764=EDGE_CURVE('',#41829,#41828,#33916,.T.);
#53765=EDGE_CURVE('',#41830,#41829,#33917,.T.);
#53766=EDGE_CURVE('',#41830,#41825,#22607,.T.);
#53767=EDGE_CURVE('',#41828,#41831,#22608,.T.);
#53768=EDGE_CURVE('',#41831,#41832,#33918,.T.);
#53769=EDGE_CURVE('',#41832,#41829,#22609,.T.);
#53770=EDGE_CURVE('',#40826,#41814,#33919,.T.);
#53771=EDGE_CURVE('',#41813,#40827,#33920,.T.);
#53772=EDGE_CURVE('',#41831,#40623,#1610,.T.);
#53773=EDGE_CURVE('',#40622,#41832,#1611,.T.);
#53774=EDGE_CURVE('',#41823,#41826,#1612,.T.);
#53775=EDGE_CURVE('',#41825,#41824,#1613,.T.);
#53776=EDGE_CURVE('',#41819,#41822,#1614,.T.);
#53777=EDGE_CURVE('',#41821,#41820,#1615,.T.);
#53778=EDGE_CURVE('',#41833,#41834,#33921,.T.);
#53779=EDGE_CURVE('',#41834,#41835,#22610,.T.);
#53780=EDGE_CURVE('',#41836,#41835,#33922,.T.);
#53781=EDGE_CURVE('',#41837,#41836,#33923,.T.);
#53782=EDGE_CURVE('',#41838,#41837,#33924,.T.);
#53783=EDGE_CURVE('',#41838,#41833,#22611,.T.);
#53784=EDGE_CURVE('',#41836,#41839,#22612,.T.);
#53785=EDGE_CURVE('',#41839,#41840,#33925,.T.);
#53786=EDGE_CURVE('',#41840,#41837,#22613,.T.);
#53787=EDGE_CURVE('',#41841,#41842,#33926,.T.);
#53788=EDGE_CURVE('',#41842,#41843,#22614,.T.);
#53789=EDGE_CURVE('',#41843,#41844,#33927,.T.);
#53790=EDGE_CURVE('',#41844,#41841,#22615,.T.);
#53791=EDGE_CURVE('',#41845,#41846,#33928,.T.);
#53792=EDGE_CURVE('',#41846,#41847,#22616,.T.);
#53793=EDGE_CURVE('',#41848,#41847,#33929,.T.);
#53794=EDGE_CURVE('',#41849,#41848,#33930,.T.);
#53795=EDGE_CURVE('',#41850,#41849,#33931,.T.);
#53796=EDGE_CURVE('',#41850,#41845,#22617,.T.);
#53797=EDGE_CURVE('',#41848,#41851,#22618,.T.);
#53798=EDGE_CURVE('',#41851,#41852,#33932,.T.);
#53799=EDGE_CURVE('',#41852,#41849,#22619,.T.);
#53800=EDGE_CURVE('',#40832,#41834,#33933,.T.);
#53801=EDGE_CURVE('',#41833,#40833,#33934,.T.);
#53802=EDGE_CURVE('',#41851,#40617,#1616,.T.);
#53803=EDGE_CURVE('',#40616,#41852,#1617,.T.);
#53804=EDGE_CURVE('',#41843,#41846,#1618,.T.);
#53805=EDGE_CURVE('',#41845,#41844,#1619,.T.);
#53806=EDGE_CURVE('',#41839,#41842,#1620,.T.);
#53807=EDGE_CURVE('',#41841,#41840,#1621,.T.);
#53808=EDGE_CURVE('',#41853,#41854,#33935,.T.);
#53809=EDGE_CURVE('',#41854,#41855,#22620,.T.);
#53810=EDGE_CURVE('',#41856,#41855,#33936,.T.);
#53811=EDGE_CURVE('',#41857,#41856,#33937,.T.);
#53812=EDGE_CURVE('',#41858,#41857,#33938,.T.);
#53813=EDGE_CURVE('',#41858,#41853,#22621,.T.);
#53814=EDGE_CURVE('',#41856,#41859,#22622,.T.);
#53815=EDGE_CURVE('',#41859,#41860,#33939,.T.);
#53816=EDGE_CURVE('',#41860,#41857,#22623,.T.);
#53817=EDGE_CURVE('',#41861,#41862,#33940,.T.);
#53818=EDGE_CURVE('',#41862,#41863,#22624,.T.);
#53819=EDGE_CURVE('',#41863,#41864,#33941,.T.);
#53820=EDGE_CURVE('',#41864,#41861,#22625,.T.);
#53821=EDGE_CURVE('',#41865,#41866,#33942,.T.);
#53822=EDGE_CURVE('',#41866,#41867,#22626,.T.);
#53823=EDGE_CURVE('',#41868,#41867,#33943,.T.);
#53824=EDGE_CURVE('',#41869,#41868,#33944,.T.);
#53825=EDGE_CURVE('',#41870,#41869,#33945,.T.);
#53826=EDGE_CURVE('',#41870,#41865,#22627,.T.);
#53827=EDGE_CURVE('',#41868,#41871,#22628,.T.);
#53828=EDGE_CURVE('',#41871,#41872,#33946,.T.);
#53829=EDGE_CURVE('',#41872,#41869,#22629,.T.);
#53830=EDGE_CURVE('',#40838,#41854,#33947,.T.);
#53831=EDGE_CURVE('',#41853,#40839,#33948,.T.);
#53832=EDGE_CURVE('',#41871,#40611,#1622,.T.);
#53833=EDGE_CURVE('',#40610,#41872,#1623,.T.);
#53834=EDGE_CURVE('',#41863,#41866,#1624,.T.);
#53835=EDGE_CURVE('',#41865,#41864,#1625,.T.);
#53836=EDGE_CURVE('',#41859,#41862,#1626,.T.);
#53837=EDGE_CURVE('',#41861,#41860,#1627,.T.);
#53838=EDGE_CURVE('',#41873,#41874,#33949,.T.);
#53839=EDGE_CURVE('',#41874,#41875,#22630,.T.);
#53840=EDGE_CURVE('',#41876,#41875,#33950,.T.);
#53841=EDGE_CURVE('',#41877,#41876,#33951,.T.);
#53842=EDGE_CURVE('',#41878,#41877,#33952,.T.);
#53843=EDGE_CURVE('',#41878,#41873,#22631,.T.);
#53844=EDGE_CURVE('',#41876,#41879,#22632,.T.);
#53845=EDGE_CURVE('',#41879,#41880,#33953,.T.);
#53846=EDGE_CURVE('',#41880,#41877,#22633,.T.);
#53847=EDGE_CURVE('',#41881,#41882,#33954,.T.);
#53848=EDGE_CURVE('',#41882,#41883,#22634,.T.);
#53849=EDGE_CURVE('',#41883,#41884,#33955,.T.);
#53850=EDGE_CURVE('',#41884,#41881,#22635,.T.);
#53851=EDGE_CURVE('',#41885,#41886,#33956,.T.);
#53852=EDGE_CURVE('',#41886,#41887,#22636,.T.);
#53853=EDGE_CURVE('',#41888,#41887,#33957,.T.);
#53854=EDGE_CURVE('',#41889,#41888,#33958,.T.);
#53855=EDGE_CURVE('',#41890,#41889,#33959,.T.);
#53856=EDGE_CURVE('',#41890,#41885,#22637,.T.);
#53857=EDGE_CURVE('',#41888,#41891,#22638,.T.);
#53858=EDGE_CURVE('',#41891,#41892,#33960,.T.);
#53859=EDGE_CURVE('',#41892,#41889,#22639,.T.);
#53860=EDGE_CURVE('',#40844,#41874,#33961,.T.);
#53861=EDGE_CURVE('',#41873,#40845,#33962,.T.);
#53862=EDGE_CURVE('',#41891,#40605,#1628,.T.);
#53863=EDGE_CURVE('',#40604,#41892,#1629,.T.);
#53864=EDGE_CURVE('',#41883,#41886,#1630,.T.);
#53865=EDGE_CURVE('',#41885,#41884,#1631,.T.);
#53866=EDGE_CURVE('',#41879,#41882,#1632,.T.);
#53867=EDGE_CURVE('',#41881,#41880,#1633,.T.);
#53868=EDGE_CURVE('',#41893,#41894,#33963,.T.);
#53869=EDGE_CURVE('',#41894,#41895,#22640,.T.);
#53870=EDGE_CURVE('',#41896,#41895,#33964,.T.);
#53871=EDGE_CURVE('',#41897,#41896,#33965,.T.);
#53872=EDGE_CURVE('',#41898,#41897,#33966,.T.);
#53873=EDGE_CURVE('',#41898,#41893,#22641,.T.);
#53874=EDGE_CURVE('',#41896,#41899,#22642,.T.);
#53875=EDGE_CURVE('',#41899,#41900,#33967,.T.);
#53876=EDGE_CURVE('',#41900,#41897,#22643,.T.);
#53877=EDGE_CURVE('',#41901,#41902,#33968,.T.);
#53878=EDGE_CURVE('',#41902,#41903,#22644,.T.);
#53879=EDGE_CURVE('',#41903,#41904,#33969,.T.);
#53880=EDGE_CURVE('',#41904,#41901,#22645,.T.);
#53881=EDGE_CURVE('',#41905,#41906,#33970,.T.);
#53882=EDGE_CURVE('',#41906,#41907,#22646,.T.);
#53883=EDGE_CURVE('',#41908,#41907,#33971,.T.);
#53884=EDGE_CURVE('',#41909,#41908,#33972,.T.);
#53885=EDGE_CURVE('',#41910,#41909,#33973,.T.);
#53886=EDGE_CURVE('',#41910,#41905,#22647,.T.);
#53887=EDGE_CURVE('',#41908,#41911,#22648,.T.);
#53888=EDGE_CURVE('',#41911,#41912,#33974,.T.);
#53889=EDGE_CURVE('',#41912,#41909,#22649,.T.);
#53890=EDGE_CURVE('',#40850,#41894,#33975,.T.);
#53891=EDGE_CURVE('',#41893,#40851,#33976,.T.);
#53892=EDGE_CURVE('',#41911,#40599,#1634,.T.);
#53893=EDGE_CURVE('',#40598,#41912,#1635,.T.);
#53894=EDGE_CURVE('',#41903,#41906,#1636,.T.);
#53895=EDGE_CURVE('',#41905,#41904,#1637,.T.);
#53896=EDGE_CURVE('',#41899,#41902,#1638,.T.);
#53897=EDGE_CURVE('',#41901,#41900,#1639,.T.);
#53898=EDGE_CURVE('',#41913,#41914,#33977,.T.);
#53899=EDGE_CURVE('',#41914,#41915,#22650,.T.);
#53900=EDGE_CURVE('',#41916,#41915,#33978,.T.);
#53901=EDGE_CURVE('',#41917,#41916,#33979,.T.);
#53902=EDGE_CURVE('',#41918,#41917,#33980,.T.);
#53903=EDGE_CURVE('',#41918,#41913,#22651,.T.);
#53904=EDGE_CURVE('',#41916,#41919,#22652,.T.);
#53905=EDGE_CURVE('',#41919,#41920,#33981,.T.);
#53906=EDGE_CURVE('',#41920,#41917,#22653,.T.);
#53907=EDGE_CURVE('',#41921,#41922,#33982,.T.);
#53908=EDGE_CURVE('',#41922,#41923,#22654,.T.);
#53909=EDGE_CURVE('',#41923,#41924,#33983,.T.);
#53910=EDGE_CURVE('',#41924,#41921,#22655,.T.);
#53911=EDGE_CURVE('',#41925,#41926,#33984,.T.);
#53912=EDGE_CURVE('',#41926,#41927,#22656,.T.);
#53913=EDGE_CURVE('',#41928,#41927,#33985,.T.);
#53914=EDGE_CURVE('',#41929,#41928,#33986,.T.);
#53915=EDGE_CURVE('',#41930,#41929,#33987,.T.);
#53916=EDGE_CURVE('',#41930,#41925,#22657,.T.);
#53917=EDGE_CURVE('',#41928,#41931,#22658,.T.);
#53918=EDGE_CURVE('',#41931,#41932,#33988,.T.);
#53919=EDGE_CURVE('',#41932,#41929,#22659,.T.);
#53920=EDGE_CURVE('',#40856,#41914,#33989,.T.);
#53921=EDGE_CURVE('',#41913,#40857,#33990,.T.);
#53922=EDGE_CURVE('',#41931,#40593,#1640,.T.);
#53923=EDGE_CURVE('',#40592,#41932,#1641,.T.);
#53924=EDGE_CURVE('',#41923,#41926,#1642,.T.);
#53925=EDGE_CURVE('',#41925,#41924,#1643,.T.);
#53926=EDGE_CURVE('',#41919,#41922,#1644,.T.);
#53927=EDGE_CURVE('',#41921,#41920,#1645,.T.);
#53928=EDGE_CURVE('',#41933,#41934,#33991,.T.);
#53929=EDGE_CURVE('',#41934,#41935,#22660,.T.);
#53930=EDGE_CURVE('',#41936,#41935,#33992,.T.);
#53931=EDGE_CURVE('',#41937,#41936,#33993,.T.);
#53932=EDGE_CURVE('',#41938,#41937,#33994,.T.);
#53933=EDGE_CURVE('',#41938,#41933,#22661,.T.);
#53934=EDGE_CURVE('',#41936,#41939,#22662,.T.);
#53935=EDGE_CURVE('',#41939,#41940,#33995,.T.);
#53936=EDGE_CURVE('',#41940,#41937,#22663,.T.);
#53937=EDGE_CURVE('',#41941,#41942,#33996,.T.);
#53938=EDGE_CURVE('',#41942,#41943,#22664,.T.);
#53939=EDGE_CURVE('',#41943,#41944,#33997,.T.);
#53940=EDGE_CURVE('',#41944,#41941,#22665,.T.);
#53941=EDGE_CURVE('',#41945,#41946,#33998,.T.);
#53942=EDGE_CURVE('',#41946,#41947,#22666,.T.);
#53943=EDGE_CURVE('',#41948,#41947,#33999,.T.);
#53944=EDGE_CURVE('',#41949,#41948,#34000,.T.);
#53945=EDGE_CURVE('',#41950,#41949,#34001,.T.);
#53946=EDGE_CURVE('',#41950,#41945,#22667,.T.);
#53947=EDGE_CURVE('',#41948,#41951,#22668,.T.);
#53948=EDGE_CURVE('',#41951,#41952,#34002,.T.);
#53949=EDGE_CURVE('',#41952,#41949,#22669,.T.);
#53950=EDGE_CURVE('',#40862,#41934,#34003,.T.);
#53951=EDGE_CURVE('',#41933,#40863,#34004,.T.);
#53952=EDGE_CURVE('',#41951,#40587,#1646,.T.);
#53953=EDGE_CURVE('',#40586,#41952,#1647,.T.);
#53954=EDGE_CURVE('',#41943,#41946,#1648,.T.);
#53955=EDGE_CURVE('',#41945,#41944,#1649,.T.);
#53956=EDGE_CURVE('',#41939,#41942,#1650,.T.);
#53957=EDGE_CURVE('',#41941,#41940,#1651,.T.);
#53958=EDGE_CURVE('',#41953,#41954,#34005,.T.);
#53959=EDGE_CURVE('',#41954,#41955,#22670,.T.);
#53960=EDGE_CURVE('',#41956,#41955,#34006,.T.);
#53961=EDGE_CURVE('',#41957,#41956,#34007,.T.);
#53962=EDGE_CURVE('',#41958,#41957,#34008,.T.);
#53963=EDGE_CURVE('',#41958,#41953,#22671,.T.);
#53964=EDGE_CURVE('',#41956,#41959,#22672,.T.);
#53965=EDGE_CURVE('',#41959,#41960,#34009,.T.);
#53966=EDGE_CURVE('',#41960,#41957,#22673,.T.);
#53967=EDGE_CURVE('',#41961,#41962,#34010,.T.);
#53968=EDGE_CURVE('',#41962,#41963,#22674,.T.);
#53969=EDGE_CURVE('',#41963,#41964,#34011,.T.);
#53970=EDGE_CURVE('',#41964,#41961,#22675,.T.);
#53971=EDGE_CURVE('',#41965,#41966,#34012,.T.);
#53972=EDGE_CURVE('',#41966,#41967,#22676,.T.);
#53973=EDGE_CURVE('',#41968,#41967,#34013,.T.);
#53974=EDGE_CURVE('',#41969,#41968,#34014,.T.);
#53975=EDGE_CURVE('',#41970,#41969,#34015,.T.);
#53976=EDGE_CURVE('',#41970,#41965,#22677,.T.);
#53977=EDGE_CURVE('',#41968,#41971,#22678,.T.);
#53978=EDGE_CURVE('',#41971,#41972,#34016,.T.);
#53979=EDGE_CURVE('',#41972,#41969,#22679,.T.);
#53980=EDGE_CURVE('',#40868,#41954,#34017,.T.);
#53981=EDGE_CURVE('',#41953,#40869,#34018,.T.);
#53982=EDGE_CURVE('',#41971,#40581,#1652,.T.);
#53983=EDGE_CURVE('',#40580,#41972,#1653,.T.);
#53984=EDGE_CURVE('',#41963,#41966,#1654,.T.);
#53985=EDGE_CURVE('',#41965,#41964,#1655,.T.);
#53986=EDGE_CURVE('',#41959,#41962,#1656,.T.);
#53987=EDGE_CURVE('',#41961,#41960,#1657,.T.);
#53988=EDGE_CURVE('',#41973,#41974,#34019,.T.);
#53989=EDGE_CURVE('',#41974,#41975,#22680,.T.);
#53990=EDGE_CURVE('',#41976,#41975,#34020,.T.);
#53991=EDGE_CURVE('',#41977,#41976,#34021,.T.);
#53992=EDGE_CURVE('',#41978,#41977,#34022,.T.);
#53993=EDGE_CURVE('',#41978,#41973,#22681,.T.);
#53994=EDGE_CURVE('',#41976,#41979,#22682,.T.);
#53995=EDGE_CURVE('',#41979,#41980,#34023,.T.);
#53996=EDGE_CURVE('',#41980,#41977,#22683,.T.);
#53997=EDGE_CURVE('',#41981,#41982,#34024,.T.);
#53998=EDGE_CURVE('',#41982,#41983,#22684,.T.);
#53999=EDGE_CURVE('',#41983,#41984,#34025,.T.);
#54000=EDGE_CURVE('',#41984,#41981,#22685,.T.);
#54001=EDGE_CURVE('',#41985,#41986,#34026,.T.);
#54002=EDGE_CURVE('',#41986,#41987,#22686,.T.);
#54003=EDGE_CURVE('',#41988,#41987,#34027,.T.);
#54004=EDGE_CURVE('',#41989,#41988,#34028,.T.);
#54005=EDGE_CURVE('',#41990,#41989,#34029,.T.);
#54006=EDGE_CURVE('',#41990,#41985,#22687,.T.);
#54007=EDGE_CURVE('',#41988,#41991,#22688,.T.);
#54008=EDGE_CURVE('',#41991,#41992,#34030,.T.);
#54009=EDGE_CURVE('',#41992,#41989,#22689,.T.);
#54010=EDGE_CURVE('',#40874,#41974,#34031,.T.);
#54011=EDGE_CURVE('',#41973,#40875,#34032,.T.);
#54012=EDGE_CURVE('',#41991,#40575,#1658,.T.);
#54013=EDGE_CURVE('',#40574,#41992,#1659,.T.);
#54014=EDGE_CURVE('',#41983,#41986,#1660,.T.);
#54015=EDGE_CURVE('',#41985,#41984,#1661,.T.);
#54016=EDGE_CURVE('',#41979,#41982,#1662,.T.);
#54017=EDGE_CURVE('',#41981,#41980,#1663,.T.);
#54018=EDGE_CURVE('',#41993,#41994,#34033,.T.);
#54019=EDGE_CURVE('',#41994,#41995,#22690,.T.);
#54020=EDGE_CURVE('',#41996,#41995,#34034,.T.);
#54021=EDGE_CURVE('',#41997,#41996,#34035,.T.);
#54022=EDGE_CURVE('',#41998,#41997,#34036,.T.);
#54023=EDGE_CURVE('',#41998,#41993,#22691,.T.);
#54024=EDGE_CURVE('',#41996,#41999,#22692,.T.);
#54025=EDGE_CURVE('',#41999,#42000,#34037,.T.);
#54026=EDGE_CURVE('',#42000,#41997,#22693,.T.);
#54027=EDGE_CURVE('',#42001,#42002,#34038,.T.);
#54028=EDGE_CURVE('',#42002,#42003,#22694,.T.);
#54029=EDGE_CURVE('',#42003,#42004,#34039,.T.);
#54030=EDGE_CURVE('',#42004,#42001,#22695,.T.);
#54031=EDGE_CURVE('',#42005,#42006,#34040,.T.);
#54032=EDGE_CURVE('',#42006,#42007,#22696,.T.);
#54033=EDGE_CURVE('',#42008,#42007,#34041,.T.);
#54034=EDGE_CURVE('',#42009,#42008,#34042,.T.);
#54035=EDGE_CURVE('',#42010,#42009,#34043,.T.);
#54036=EDGE_CURVE('',#42010,#42005,#22697,.T.);
#54037=EDGE_CURVE('',#42008,#42011,#22698,.T.);
#54038=EDGE_CURVE('',#42011,#42012,#34044,.T.);
#54039=EDGE_CURVE('',#42012,#42009,#22699,.T.);
#54040=EDGE_CURVE('',#40880,#41994,#34045,.T.);
#54041=EDGE_CURVE('',#41993,#40881,#34046,.T.);
#54042=EDGE_CURVE('',#42011,#40569,#1664,.T.);
#54043=EDGE_CURVE('',#40568,#42012,#1665,.T.);
#54044=EDGE_CURVE('',#42003,#42006,#1666,.T.);
#54045=EDGE_CURVE('',#42005,#42004,#1667,.T.);
#54046=EDGE_CURVE('',#41999,#42002,#1668,.T.);
#54047=EDGE_CURVE('',#42001,#42000,#1669,.T.);
#54048=EDGE_CURVE('',#42013,#42014,#34047,.T.);
#54049=EDGE_CURVE('',#42014,#42015,#22700,.T.);
#54050=EDGE_CURVE('',#42016,#42015,#34048,.T.);
#54051=EDGE_CURVE('',#42017,#42016,#34049,.T.);
#54052=EDGE_CURVE('',#42018,#42017,#34050,.T.);
#54053=EDGE_CURVE('',#42018,#42013,#22701,.T.);
#54054=EDGE_CURVE('',#42016,#42019,#22702,.T.);
#54055=EDGE_CURVE('',#42019,#42020,#34051,.T.);
#54056=EDGE_CURVE('',#42020,#42017,#22703,.T.);
#54057=EDGE_CURVE('',#42021,#42022,#34052,.T.);
#54058=EDGE_CURVE('',#42022,#42023,#22704,.T.);
#54059=EDGE_CURVE('',#42023,#42024,#34053,.T.);
#54060=EDGE_CURVE('',#42024,#42021,#22705,.T.);
#54061=EDGE_CURVE('',#42025,#42026,#34054,.T.);
#54062=EDGE_CURVE('',#42026,#42027,#22706,.T.);
#54063=EDGE_CURVE('',#42028,#42027,#34055,.T.);
#54064=EDGE_CURVE('',#42029,#42028,#34056,.T.);
#54065=EDGE_CURVE('',#42030,#42029,#34057,.T.);
#54066=EDGE_CURVE('',#42030,#42025,#22707,.T.);
#54067=EDGE_CURVE('',#42028,#42031,#22708,.T.);
#54068=EDGE_CURVE('',#42031,#42032,#34058,.T.);
#54069=EDGE_CURVE('',#42032,#42029,#22709,.T.);
#54070=EDGE_CURVE('',#40886,#42014,#34059,.T.);
#54071=EDGE_CURVE('',#42013,#40887,#34060,.T.);
#54072=EDGE_CURVE('',#42031,#40563,#1670,.T.);
#54073=EDGE_CURVE('',#40562,#42032,#1671,.T.);
#54074=EDGE_CURVE('',#42023,#42026,#1672,.T.);
#54075=EDGE_CURVE('',#42025,#42024,#1673,.T.);
#54076=EDGE_CURVE('',#42019,#42022,#1674,.T.);
#54077=EDGE_CURVE('',#42021,#42020,#1675,.T.);
#54078=EDGE_CURVE('',#42033,#42034,#34061,.T.);
#54079=EDGE_CURVE('',#42034,#42035,#22710,.T.);
#54080=EDGE_CURVE('',#42036,#42035,#34062,.T.);
#54081=EDGE_CURVE('',#42037,#42036,#34063,.T.);
#54082=EDGE_CURVE('',#42038,#42037,#34064,.T.);
#54083=EDGE_CURVE('',#42038,#42033,#22711,.T.);
#54084=EDGE_CURVE('',#42036,#42039,#22712,.T.);
#54085=EDGE_CURVE('',#42039,#42040,#34065,.T.);
#54086=EDGE_CURVE('',#42040,#42037,#22713,.T.);
#54087=EDGE_CURVE('',#42041,#42042,#34066,.T.);
#54088=EDGE_CURVE('',#42042,#42043,#22714,.T.);
#54089=EDGE_CURVE('',#42043,#42044,#34067,.T.);
#54090=EDGE_CURVE('',#42044,#42041,#22715,.T.);
#54091=EDGE_CURVE('',#42045,#42046,#34068,.T.);
#54092=EDGE_CURVE('',#42046,#42047,#22716,.T.);
#54093=EDGE_CURVE('',#42048,#42047,#34069,.T.);
#54094=EDGE_CURVE('',#42049,#42048,#34070,.T.);
#54095=EDGE_CURVE('',#42050,#42049,#34071,.T.);
#54096=EDGE_CURVE('',#42050,#42045,#22717,.T.);
#54097=EDGE_CURVE('',#42048,#42051,#22718,.T.);
#54098=EDGE_CURVE('',#42051,#42052,#34072,.T.);
#54099=EDGE_CURVE('',#42052,#42049,#22719,.T.);
#54100=EDGE_CURVE('',#40892,#42034,#34073,.T.);
#54101=EDGE_CURVE('',#42033,#40893,#34074,.T.);
#54102=EDGE_CURVE('',#42051,#40557,#1676,.T.);
#54103=EDGE_CURVE('',#40556,#42052,#1677,.T.);
#54104=EDGE_CURVE('',#42043,#42046,#1678,.T.);
#54105=EDGE_CURVE('',#42045,#42044,#1679,.T.);
#54106=EDGE_CURVE('',#42039,#42042,#1680,.T.);
#54107=EDGE_CURVE('',#42041,#42040,#1681,.T.);
#54108=EDGE_CURVE('',#42053,#42054,#34075,.T.);
#54109=EDGE_CURVE('',#42054,#42055,#22720,.T.);
#54110=EDGE_CURVE('',#42056,#42055,#34076,.T.);
#54111=EDGE_CURVE('',#42057,#42056,#34077,.T.);
#54112=EDGE_CURVE('',#42058,#42057,#34078,.T.);
#54113=EDGE_CURVE('',#42058,#42053,#22721,.T.);
#54114=EDGE_CURVE('',#42056,#42059,#22722,.T.);
#54115=EDGE_CURVE('',#42059,#42060,#34079,.T.);
#54116=EDGE_CURVE('',#42060,#42057,#22723,.T.);
#54117=EDGE_CURVE('',#42061,#42062,#34080,.T.);
#54118=EDGE_CURVE('',#42062,#42063,#22724,.T.);
#54119=EDGE_CURVE('',#42063,#42064,#34081,.T.);
#54120=EDGE_CURVE('',#42064,#42061,#22725,.T.);
#54121=EDGE_CURVE('',#42065,#42066,#34082,.T.);
#54122=EDGE_CURVE('',#42066,#42067,#22726,.T.);
#54123=EDGE_CURVE('',#42068,#42067,#34083,.T.);
#54124=EDGE_CURVE('',#42069,#42068,#34084,.T.);
#54125=EDGE_CURVE('',#42070,#42069,#34085,.T.);
#54126=EDGE_CURVE('',#42070,#42065,#22727,.T.);
#54127=EDGE_CURVE('',#42068,#42071,#22728,.T.);
#54128=EDGE_CURVE('',#42071,#42072,#34086,.T.);
#54129=EDGE_CURVE('',#42072,#42069,#22729,.T.);
#54130=EDGE_CURVE('',#40898,#42054,#34087,.T.);
#54131=EDGE_CURVE('',#42053,#40899,#34088,.T.);
#54132=EDGE_CURVE('',#42071,#40551,#1682,.T.);
#54133=EDGE_CURVE('',#40550,#42072,#1683,.T.);
#54134=EDGE_CURVE('',#42063,#42066,#1684,.T.);
#54135=EDGE_CURVE('',#42065,#42064,#1685,.T.);
#54136=EDGE_CURVE('',#42059,#42062,#1686,.T.);
#54137=EDGE_CURVE('',#42061,#42060,#1687,.T.);
#54138=EDGE_CURVE('',#42073,#42074,#34089,.T.);
#54139=EDGE_CURVE('',#42074,#42075,#22730,.T.);
#54140=EDGE_CURVE('',#42076,#42075,#34090,.T.);
#54141=EDGE_CURVE('',#42077,#42076,#34091,.T.);
#54142=EDGE_CURVE('',#42078,#42077,#34092,.T.);
#54143=EDGE_CURVE('',#42078,#42073,#22731,.T.);
#54144=EDGE_CURVE('',#42076,#42079,#22732,.T.);
#54145=EDGE_CURVE('',#42079,#42080,#34093,.T.);
#54146=EDGE_CURVE('',#42080,#42077,#22733,.T.);
#54147=EDGE_CURVE('',#42081,#42082,#34094,.T.);
#54148=EDGE_CURVE('',#42082,#42083,#22734,.T.);
#54149=EDGE_CURVE('',#42083,#42084,#34095,.T.);
#54150=EDGE_CURVE('',#42084,#42081,#22735,.T.);
#54151=EDGE_CURVE('',#42085,#42086,#34096,.T.);
#54152=EDGE_CURVE('',#42086,#42087,#22736,.T.);
#54153=EDGE_CURVE('',#42088,#42087,#34097,.T.);
#54154=EDGE_CURVE('',#42089,#42088,#34098,.T.);
#54155=EDGE_CURVE('',#42090,#42089,#34099,.T.);
#54156=EDGE_CURVE('',#42090,#42085,#22737,.T.);
#54157=EDGE_CURVE('',#42088,#42091,#22738,.T.);
#54158=EDGE_CURVE('',#42091,#42092,#34100,.T.);
#54159=EDGE_CURVE('',#42092,#42089,#22739,.T.);
#54160=EDGE_CURVE('',#40904,#42074,#34101,.T.);
#54161=EDGE_CURVE('',#42073,#40905,#34102,.T.);
#54162=EDGE_CURVE('',#42091,#40545,#1688,.T.);
#54163=EDGE_CURVE('',#40544,#42092,#1689,.T.);
#54164=EDGE_CURVE('',#42083,#42086,#1690,.T.);
#54165=EDGE_CURVE('',#42085,#42084,#1691,.T.);
#54166=EDGE_CURVE('',#42079,#42082,#1692,.T.);
#54167=EDGE_CURVE('',#42081,#42080,#1693,.T.);
#54168=EDGE_CURVE('',#42093,#42094,#34103,.T.);
#54169=EDGE_CURVE('',#42094,#42095,#22740,.T.);
#54170=EDGE_CURVE('',#42096,#42095,#34104,.T.);
#54171=EDGE_CURVE('',#42097,#42096,#34105,.T.);
#54172=EDGE_CURVE('',#42098,#42097,#34106,.T.);
#54173=EDGE_CURVE('',#42098,#42093,#22741,.T.);
#54174=EDGE_CURVE('',#42096,#42099,#22742,.T.);
#54175=EDGE_CURVE('',#42099,#42100,#34107,.T.);
#54176=EDGE_CURVE('',#42100,#42097,#22743,.T.);
#54177=EDGE_CURVE('',#42101,#42102,#34108,.T.);
#54178=EDGE_CURVE('',#42102,#42103,#22744,.T.);
#54179=EDGE_CURVE('',#42103,#42104,#34109,.T.);
#54180=EDGE_CURVE('',#42104,#42101,#22745,.T.);
#54181=EDGE_CURVE('',#42105,#42106,#34110,.T.);
#54182=EDGE_CURVE('',#42106,#42107,#22746,.T.);
#54183=EDGE_CURVE('',#42108,#42107,#34111,.T.);
#54184=EDGE_CURVE('',#42109,#42108,#34112,.T.);
#54185=EDGE_CURVE('',#42110,#42109,#34113,.T.);
#54186=EDGE_CURVE('',#42110,#42105,#22747,.T.);
#54187=EDGE_CURVE('',#42108,#42111,#22748,.T.);
#54188=EDGE_CURVE('',#42111,#42112,#34114,.T.);
#54189=EDGE_CURVE('',#42112,#42109,#22749,.T.);
#54190=EDGE_CURVE('',#40910,#42094,#34115,.T.);
#54191=EDGE_CURVE('',#42093,#40911,#34116,.T.);
#54192=EDGE_CURVE('',#42111,#40539,#1694,.T.);
#54193=EDGE_CURVE('',#40538,#42112,#1695,.T.);
#54194=EDGE_CURVE('',#42103,#42106,#1696,.T.);
#54195=EDGE_CURVE('',#42105,#42104,#1697,.T.);
#54196=EDGE_CURVE('',#42099,#42102,#1698,.T.);
#54197=EDGE_CURVE('',#42101,#42100,#1699,.T.);
#54198=EDGE_CURVE('',#42113,#42114,#34117,.T.);
#54199=EDGE_CURVE('',#42114,#42115,#22750,.T.);
#54200=EDGE_CURVE('',#42116,#42115,#34118,.T.);
#54201=EDGE_CURVE('',#42117,#42116,#34119,.T.);
#54202=EDGE_CURVE('',#42118,#42117,#34120,.T.);
#54203=EDGE_CURVE('',#42118,#42113,#22751,.T.);
#54204=EDGE_CURVE('',#42116,#42119,#22752,.T.);
#54205=EDGE_CURVE('',#42119,#42120,#34121,.T.);
#54206=EDGE_CURVE('',#42120,#42117,#22753,.T.);
#54207=EDGE_CURVE('',#42121,#42122,#34122,.T.);
#54208=EDGE_CURVE('',#42122,#42123,#22754,.T.);
#54209=EDGE_CURVE('',#42123,#42124,#34123,.T.);
#54210=EDGE_CURVE('',#42124,#42121,#22755,.T.);
#54211=EDGE_CURVE('',#42125,#42126,#34124,.T.);
#54212=EDGE_CURVE('',#42126,#42127,#22756,.T.);
#54213=EDGE_CURVE('',#42128,#42127,#34125,.T.);
#54214=EDGE_CURVE('',#42129,#42128,#34126,.T.);
#54215=EDGE_CURVE('',#42130,#42129,#34127,.T.);
#54216=EDGE_CURVE('',#42130,#42125,#22757,.T.);
#54217=EDGE_CURVE('',#42128,#42131,#22758,.T.);
#54218=EDGE_CURVE('',#42131,#42132,#34128,.T.);
#54219=EDGE_CURVE('',#42132,#42129,#22759,.T.);
#54220=EDGE_CURVE('',#40916,#42114,#34129,.T.);
#54221=EDGE_CURVE('',#42113,#40917,#34130,.T.);
#54222=EDGE_CURVE('',#42131,#40533,#1700,.T.);
#54223=EDGE_CURVE('',#40532,#42132,#1701,.T.);
#54224=EDGE_CURVE('',#42123,#42126,#1702,.T.);
#54225=EDGE_CURVE('',#42125,#42124,#1703,.T.);
#54226=EDGE_CURVE('',#42119,#42122,#1704,.T.);
#54227=EDGE_CURVE('',#42121,#42120,#1705,.T.);
#54228=EDGE_CURVE('',#42133,#42134,#34131,.T.);
#54229=EDGE_CURVE('',#42134,#42135,#22760,.T.);
#54230=EDGE_CURVE('',#42136,#42135,#34132,.T.);
#54231=EDGE_CURVE('',#42137,#42136,#34133,.T.);
#54232=EDGE_CURVE('',#42138,#42137,#34134,.T.);
#54233=EDGE_CURVE('',#42138,#42133,#22761,.T.);
#54234=EDGE_CURVE('',#42136,#42139,#22762,.T.);
#54235=EDGE_CURVE('',#42139,#42140,#34135,.T.);
#54236=EDGE_CURVE('',#42140,#42137,#22763,.T.);
#54237=EDGE_CURVE('',#42141,#42142,#34136,.T.);
#54238=EDGE_CURVE('',#42142,#42143,#22764,.T.);
#54239=EDGE_CURVE('',#42143,#42144,#34137,.T.);
#54240=EDGE_CURVE('',#42144,#42141,#22765,.T.);
#54241=EDGE_CURVE('',#42145,#42146,#34138,.T.);
#54242=EDGE_CURVE('',#42146,#42147,#22766,.T.);
#54243=EDGE_CURVE('',#42148,#42147,#34139,.T.);
#54244=EDGE_CURVE('',#42149,#42148,#34140,.T.);
#54245=EDGE_CURVE('',#42150,#42149,#34141,.T.);
#54246=EDGE_CURVE('',#42150,#42145,#22767,.T.);
#54247=EDGE_CURVE('',#42148,#42151,#22768,.T.);
#54248=EDGE_CURVE('',#42151,#42152,#34142,.T.);
#54249=EDGE_CURVE('',#42152,#42149,#22769,.T.);
#54250=EDGE_CURVE('',#40922,#42134,#34143,.T.);
#54251=EDGE_CURVE('',#42133,#40923,#34144,.T.);
#54252=EDGE_CURVE('',#42151,#40527,#1706,.T.);
#54253=EDGE_CURVE('',#40526,#42152,#1707,.T.);
#54254=EDGE_CURVE('',#42143,#42146,#1708,.T.);
#54255=EDGE_CURVE('',#42145,#42144,#1709,.T.);
#54256=EDGE_CURVE('',#42139,#42142,#1710,.T.);
#54257=EDGE_CURVE('',#42141,#42140,#1711,.T.);
#54258=EDGE_CURVE('',#42153,#42154,#34145,.T.);
#54259=EDGE_CURVE('',#42154,#42155,#22770,.T.);
#54260=EDGE_CURVE('',#42156,#42155,#34146,.T.);
#54261=EDGE_CURVE('',#42157,#42156,#34147,.T.);
#54262=EDGE_CURVE('',#42158,#42157,#34148,.T.);
#54263=EDGE_CURVE('',#42158,#42153,#22771,.T.);
#54264=EDGE_CURVE('',#42156,#42159,#22772,.T.);
#54265=EDGE_CURVE('',#42159,#42160,#34149,.T.);
#54266=EDGE_CURVE('',#42160,#42157,#22773,.T.);
#54267=EDGE_CURVE('',#42161,#42162,#34150,.T.);
#54268=EDGE_CURVE('',#42162,#42163,#22774,.T.);
#54269=EDGE_CURVE('',#42163,#42164,#34151,.T.);
#54270=EDGE_CURVE('',#42164,#42161,#22775,.T.);
#54271=EDGE_CURVE('',#42165,#42166,#34152,.T.);
#54272=EDGE_CURVE('',#42166,#42167,#22776,.T.);
#54273=EDGE_CURVE('',#42168,#42167,#34153,.T.);
#54274=EDGE_CURVE('',#42169,#42168,#34154,.T.);
#54275=EDGE_CURVE('',#42170,#42169,#34155,.T.);
#54276=EDGE_CURVE('',#42170,#42165,#22777,.T.);
#54277=EDGE_CURVE('',#42168,#42171,#22778,.T.);
#54278=EDGE_CURVE('',#42171,#42172,#34156,.T.);
#54279=EDGE_CURVE('',#42172,#42169,#22779,.T.);
#54280=EDGE_CURVE('',#40928,#42154,#34157,.T.);
#54281=EDGE_CURVE('',#42153,#40929,#34158,.T.);
#54282=EDGE_CURVE('',#42171,#40521,#1712,.T.);
#54283=EDGE_CURVE('',#40520,#42172,#1713,.T.);
#54284=EDGE_CURVE('',#42163,#42166,#1714,.T.);
#54285=EDGE_CURVE('',#42165,#42164,#1715,.T.);
#54286=EDGE_CURVE('',#42159,#42162,#1716,.T.);
#54287=EDGE_CURVE('',#42161,#42160,#1717,.T.);
#54288=EDGE_CURVE('',#42173,#42174,#34159,.T.);
#54289=EDGE_CURVE('',#42174,#42175,#22780,.T.);
#54290=EDGE_CURVE('',#42176,#42175,#34160,.T.);
#54291=EDGE_CURVE('',#42177,#42176,#34161,.T.);
#54292=EDGE_CURVE('',#42178,#42177,#34162,.T.);
#54293=EDGE_CURVE('',#42178,#42173,#22781,.T.);
#54294=EDGE_CURVE('',#42176,#42179,#22782,.T.);
#54295=EDGE_CURVE('',#42179,#42180,#34163,.T.);
#54296=EDGE_CURVE('',#42180,#42177,#22783,.T.);
#54297=EDGE_CURVE('',#42181,#42182,#34164,.T.);
#54298=EDGE_CURVE('',#42182,#42183,#22784,.T.);
#54299=EDGE_CURVE('',#42183,#42184,#34165,.T.);
#54300=EDGE_CURVE('',#42184,#42181,#22785,.T.);
#54301=EDGE_CURVE('',#42185,#42186,#34166,.T.);
#54302=EDGE_CURVE('',#42186,#42187,#22786,.T.);
#54303=EDGE_CURVE('',#42188,#42187,#34167,.T.);
#54304=EDGE_CURVE('',#42189,#42188,#34168,.T.);
#54305=EDGE_CURVE('',#42190,#42189,#34169,.T.);
#54306=EDGE_CURVE('',#42190,#42185,#22787,.T.);
#54307=EDGE_CURVE('',#42188,#42191,#22788,.T.);
#54308=EDGE_CURVE('',#42191,#42192,#34170,.T.);
#54309=EDGE_CURVE('',#42192,#42189,#22789,.T.);
#54310=EDGE_CURVE('',#40934,#42174,#34171,.T.);
#54311=EDGE_CURVE('',#42173,#40935,#34172,.T.);
#54312=EDGE_CURVE('',#42191,#40515,#1718,.T.);
#54313=EDGE_CURVE('',#40514,#42192,#1719,.T.);
#54314=EDGE_CURVE('',#42183,#42186,#1720,.T.);
#54315=EDGE_CURVE('',#42185,#42184,#1721,.T.);
#54316=EDGE_CURVE('',#42179,#42182,#1722,.T.);
#54317=EDGE_CURVE('',#42181,#42180,#1723,.T.);
#54318=EDGE_CURVE('',#42193,#42194,#34173,.T.);
#54319=EDGE_CURVE('',#42194,#42195,#22790,.T.);
#54320=EDGE_CURVE('',#42196,#42195,#34174,.T.);
#54321=EDGE_CURVE('',#42197,#42196,#34175,.T.);
#54322=EDGE_CURVE('',#42198,#42197,#34176,.T.);
#54323=EDGE_CURVE('',#42198,#42193,#22791,.T.);
#54324=EDGE_CURVE('',#42196,#42199,#22792,.T.);
#54325=EDGE_CURVE('',#42199,#42200,#34177,.T.);
#54326=EDGE_CURVE('',#42200,#42197,#22793,.T.);
#54327=EDGE_CURVE('',#42201,#42202,#34178,.T.);
#54328=EDGE_CURVE('',#42202,#42203,#22794,.T.);
#54329=EDGE_CURVE('',#42203,#42204,#34179,.T.);
#54330=EDGE_CURVE('',#42204,#42201,#22795,.T.);
#54331=EDGE_CURVE('',#42205,#42206,#34180,.T.);
#54332=EDGE_CURVE('',#42206,#42207,#22796,.T.);
#54333=EDGE_CURVE('',#42208,#42207,#34181,.T.);
#54334=EDGE_CURVE('',#42209,#42208,#34182,.T.);
#54335=EDGE_CURVE('',#42210,#42209,#34183,.T.);
#54336=EDGE_CURVE('',#42210,#42205,#22797,.T.);
#54337=EDGE_CURVE('',#42208,#42211,#22798,.T.);
#54338=EDGE_CURVE('',#42211,#42212,#34184,.T.);
#54339=EDGE_CURVE('',#42212,#42209,#22799,.T.);
#54340=EDGE_CURVE('',#40940,#42194,#34185,.T.);
#54341=EDGE_CURVE('',#42193,#40941,#34186,.T.);
#54342=EDGE_CURVE('',#42211,#40509,#1724,.T.);
#54343=EDGE_CURVE('',#40508,#42212,#1725,.T.);
#54344=EDGE_CURVE('',#42203,#42206,#1726,.T.);
#54345=EDGE_CURVE('',#42205,#42204,#1727,.T.);
#54346=EDGE_CURVE('',#42199,#42202,#1728,.T.);
#54347=EDGE_CURVE('',#42201,#42200,#1729,.T.);
#54348=EDGE_CURVE('',#42213,#42214,#34187,.T.);
#54349=EDGE_CURVE('',#42214,#42215,#22800,.T.);
#54350=EDGE_CURVE('',#42216,#42215,#34188,.T.);
#54351=EDGE_CURVE('',#42217,#42216,#34189,.T.);
#54352=EDGE_CURVE('',#42218,#42217,#34190,.T.);
#54353=EDGE_CURVE('',#42218,#42213,#22801,.T.);
#54354=EDGE_CURVE('',#42216,#42219,#22802,.T.);
#54355=EDGE_CURVE('',#42219,#42220,#34191,.T.);
#54356=EDGE_CURVE('',#42220,#42217,#22803,.T.);
#54357=EDGE_CURVE('',#42221,#42222,#34192,.T.);
#54358=EDGE_CURVE('',#42222,#42223,#22804,.T.);
#54359=EDGE_CURVE('',#42223,#42224,#34193,.T.);
#54360=EDGE_CURVE('',#42224,#42221,#22805,.T.);
#54361=EDGE_CURVE('',#42225,#42226,#34194,.T.);
#54362=EDGE_CURVE('',#42226,#42227,#22806,.T.);
#54363=EDGE_CURVE('',#42228,#42227,#34195,.T.);
#54364=EDGE_CURVE('',#42229,#42228,#34196,.T.);
#54365=EDGE_CURVE('',#42230,#42229,#34197,.T.);
#54366=EDGE_CURVE('',#42230,#42225,#22807,.T.);
#54367=EDGE_CURVE('',#42228,#42231,#22808,.T.);
#54368=EDGE_CURVE('',#42231,#42232,#34198,.T.);
#54369=EDGE_CURVE('',#42232,#42229,#22809,.T.);
#54370=EDGE_CURVE('',#40946,#42214,#34199,.T.);
#54371=EDGE_CURVE('',#42213,#40947,#34200,.T.);
#54372=EDGE_CURVE('',#42231,#40503,#1730,.T.);
#54373=EDGE_CURVE('',#40502,#42232,#1731,.T.);
#54374=EDGE_CURVE('',#42223,#42226,#1732,.T.);
#54375=EDGE_CURVE('',#42225,#42224,#1733,.T.);
#54376=EDGE_CURVE('',#42219,#42222,#1734,.T.);
#54377=EDGE_CURVE('',#42221,#42220,#1735,.T.);
#54378=EDGE_CURVE('',#42233,#42234,#34201,.T.);
#54379=EDGE_CURVE('',#42234,#42235,#22810,.T.);
#54380=EDGE_CURVE('',#42236,#42235,#34202,.T.);
#54381=EDGE_CURVE('',#42237,#42236,#34203,.T.);
#54382=EDGE_CURVE('',#42238,#42237,#34204,.T.);
#54383=EDGE_CURVE('',#42238,#42233,#22811,.T.);
#54384=EDGE_CURVE('',#42236,#42239,#22812,.T.);
#54385=EDGE_CURVE('',#42239,#42240,#34205,.T.);
#54386=EDGE_CURVE('',#42240,#42237,#22813,.T.);
#54387=EDGE_CURVE('',#42241,#42242,#34206,.T.);
#54388=EDGE_CURVE('',#42242,#42243,#22814,.T.);
#54389=EDGE_CURVE('',#42243,#42244,#34207,.T.);
#54390=EDGE_CURVE('',#42244,#42241,#22815,.T.);
#54391=EDGE_CURVE('',#42245,#42246,#34208,.T.);
#54392=EDGE_CURVE('',#42246,#42247,#22816,.T.);
#54393=EDGE_CURVE('',#42248,#42247,#34209,.T.);
#54394=EDGE_CURVE('',#42249,#42248,#34210,.T.);
#54395=EDGE_CURVE('',#42250,#42249,#34211,.T.);
#54396=EDGE_CURVE('',#42250,#42245,#22817,.T.);
#54397=EDGE_CURVE('',#42248,#42251,#22818,.T.);
#54398=EDGE_CURVE('',#42251,#42252,#34212,.T.);
#54399=EDGE_CURVE('',#42252,#42249,#22819,.T.);
#54400=EDGE_CURVE('',#40952,#42234,#34213,.T.);
#54401=EDGE_CURVE('',#42233,#40953,#34214,.T.);
#54402=EDGE_CURVE('',#42251,#40497,#1736,.T.);
#54403=EDGE_CURVE('',#40496,#42252,#1737,.T.);
#54404=EDGE_CURVE('',#42243,#42246,#1738,.T.);
#54405=EDGE_CURVE('',#42245,#42244,#1739,.T.);
#54406=EDGE_CURVE('',#42239,#42242,#1740,.T.);
#54407=EDGE_CURVE('',#42241,#42240,#1741,.T.);
#54408=EDGE_CURVE('',#42253,#42254,#34215,.T.);
#54409=EDGE_CURVE('',#42254,#42255,#22820,.T.);
#54410=EDGE_CURVE('',#42256,#42255,#34216,.T.);
#54411=EDGE_CURVE('',#42257,#42256,#34217,.T.);
#54412=EDGE_CURVE('',#42258,#42257,#34218,.T.);
#54413=EDGE_CURVE('',#42258,#42253,#22821,.T.);
#54414=EDGE_CURVE('',#42256,#42259,#22822,.T.);
#54415=EDGE_CURVE('',#42259,#42260,#34219,.T.);
#54416=EDGE_CURVE('',#42260,#42257,#22823,.T.);
#54417=EDGE_CURVE('',#42261,#42262,#34220,.T.);
#54418=EDGE_CURVE('',#42262,#42263,#22824,.T.);
#54419=EDGE_CURVE('',#42263,#42264,#34221,.T.);
#54420=EDGE_CURVE('',#42264,#42261,#22825,.T.);
#54421=EDGE_CURVE('',#42265,#42266,#34222,.T.);
#54422=EDGE_CURVE('',#42266,#42267,#22826,.T.);
#54423=EDGE_CURVE('',#42268,#42267,#34223,.T.);
#54424=EDGE_CURVE('',#42269,#42268,#34224,.T.);
#54425=EDGE_CURVE('',#42270,#42269,#34225,.T.);
#54426=EDGE_CURVE('',#42270,#42265,#22827,.T.);
#54427=EDGE_CURVE('',#42268,#42271,#22828,.T.);
#54428=EDGE_CURVE('',#42271,#42272,#34226,.T.);
#54429=EDGE_CURVE('',#42272,#42269,#22829,.T.);
#54430=EDGE_CURVE('',#40958,#42254,#34227,.T.);
#54431=EDGE_CURVE('',#42253,#40959,#34228,.T.);
#54432=EDGE_CURVE('',#42271,#40491,#1742,.T.);
#54433=EDGE_CURVE('',#40490,#42272,#1743,.T.);
#54434=EDGE_CURVE('',#42263,#42266,#1744,.T.);
#54435=EDGE_CURVE('',#42265,#42264,#1745,.T.);
#54436=EDGE_CURVE('',#42259,#42262,#1746,.T.);
#54437=EDGE_CURVE('',#42261,#42260,#1747,.T.);
#54438=EDGE_CURVE('',#42273,#42274,#34229,.T.);
#54439=EDGE_CURVE('',#42274,#42275,#22830,.T.);
#54440=EDGE_CURVE('',#42276,#42275,#34230,.T.);
#54441=EDGE_CURVE('',#42277,#42276,#34231,.T.);
#54442=EDGE_CURVE('',#42278,#42277,#34232,.T.);
#54443=EDGE_CURVE('',#42278,#42273,#22831,.T.);
#54444=EDGE_CURVE('',#42276,#42279,#22832,.T.);
#54445=EDGE_CURVE('',#42279,#42280,#34233,.T.);
#54446=EDGE_CURVE('',#42280,#42277,#22833,.T.);
#54447=EDGE_CURVE('',#42281,#42282,#34234,.T.);
#54448=EDGE_CURVE('',#42282,#42283,#22834,.T.);
#54449=EDGE_CURVE('',#42283,#42284,#34235,.T.);
#54450=EDGE_CURVE('',#42284,#42281,#22835,.T.);
#54451=EDGE_CURVE('',#42285,#42286,#34236,.T.);
#54452=EDGE_CURVE('',#42286,#42287,#22836,.T.);
#54453=EDGE_CURVE('',#42288,#42287,#34237,.T.);
#54454=EDGE_CURVE('',#42289,#42288,#34238,.T.);
#54455=EDGE_CURVE('',#42290,#42289,#34239,.T.);
#54456=EDGE_CURVE('',#42290,#42285,#22837,.T.);
#54457=EDGE_CURVE('',#42288,#42291,#22838,.T.);
#54458=EDGE_CURVE('',#42291,#42292,#34240,.T.);
#54459=EDGE_CURVE('',#42292,#42289,#22839,.T.);
#54460=EDGE_CURVE('',#40964,#42274,#34241,.T.);
#54461=EDGE_CURVE('',#42273,#40965,#34242,.T.);
#54462=EDGE_CURVE('',#42291,#40485,#1748,.T.);
#54463=EDGE_CURVE('',#40484,#42292,#1749,.T.);
#54464=EDGE_CURVE('',#42283,#42286,#1750,.T.);
#54465=EDGE_CURVE('',#42285,#42284,#1751,.T.);
#54466=EDGE_CURVE('',#42279,#42282,#1752,.T.);
#54467=EDGE_CURVE('',#42281,#42280,#1753,.T.);
#54468=EDGE_CURVE('',#42293,#42294,#34243,.T.);
#54469=EDGE_CURVE('',#42294,#42295,#22840,.T.);
#54470=EDGE_CURVE('',#42296,#42295,#34244,.T.);
#54471=EDGE_CURVE('',#42297,#42296,#34245,.T.);
#54472=EDGE_CURVE('',#42298,#42297,#34246,.T.);
#54473=EDGE_CURVE('',#42298,#42293,#22841,.T.);
#54474=EDGE_CURVE('',#42296,#42299,#22842,.T.);
#54475=EDGE_CURVE('',#42299,#42300,#34247,.T.);
#54476=EDGE_CURVE('',#42300,#42297,#22843,.T.);
#54477=EDGE_CURVE('',#42301,#42302,#34248,.T.);
#54478=EDGE_CURVE('',#42302,#42303,#22844,.T.);
#54479=EDGE_CURVE('',#42303,#42304,#34249,.T.);
#54480=EDGE_CURVE('',#42304,#42301,#22845,.T.);
#54481=EDGE_CURVE('',#42305,#42306,#34250,.T.);
#54482=EDGE_CURVE('',#42306,#42307,#22846,.T.);
#54483=EDGE_CURVE('',#42308,#42307,#34251,.T.);
#54484=EDGE_CURVE('',#42309,#42308,#34252,.T.);
#54485=EDGE_CURVE('',#42310,#42309,#34253,.T.);
#54486=EDGE_CURVE('',#42310,#42305,#22847,.T.);
#54487=EDGE_CURVE('',#42308,#42311,#22848,.T.);
#54488=EDGE_CURVE('',#42311,#42312,#34254,.T.);
#54489=EDGE_CURVE('',#42312,#42309,#22849,.T.);
#54490=EDGE_CURVE('',#40970,#42294,#34255,.T.);
#54491=EDGE_CURVE('',#42293,#40971,#34256,.T.);
#54492=EDGE_CURVE('',#42311,#40479,#1754,.T.);
#54493=EDGE_CURVE('',#40478,#42312,#1755,.T.);
#54494=EDGE_CURVE('',#42303,#42306,#1756,.T.);
#54495=EDGE_CURVE('',#42305,#42304,#1757,.T.);
#54496=EDGE_CURVE('',#42299,#42302,#1758,.T.);
#54497=EDGE_CURVE('',#42301,#42300,#1759,.T.);
#54498=EDGE_CURVE('',#42313,#42314,#34257,.T.);
#54499=EDGE_CURVE('',#42314,#42315,#22850,.T.);
#54500=EDGE_CURVE('',#42316,#42315,#34258,.T.);
#54501=EDGE_CURVE('',#42317,#42316,#34259,.T.);
#54502=EDGE_CURVE('',#42318,#42317,#34260,.T.);
#54503=EDGE_CURVE('',#42318,#42313,#22851,.T.);
#54504=EDGE_CURVE('',#42316,#42319,#22852,.T.);
#54505=EDGE_CURVE('',#42319,#42320,#34261,.T.);
#54506=EDGE_CURVE('',#42320,#42317,#22853,.T.);
#54507=EDGE_CURVE('',#42321,#42322,#34262,.T.);
#54508=EDGE_CURVE('',#42322,#42323,#22854,.T.);
#54509=EDGE_CURVE('',#42323,#42324,#34263,.T.);
#54510=EDGE_CURVE('',#42324,#42321,#22855,.T.);
#54511=EDGE_CURVE('',#42325,#42326,#34264,.T.);
#54512=EDGE_CURVE('',#42326,#42327,#22856,.T.);
#54513=EDGE_CURVE('',#42328,#42327,#34265,.T.);
#54514=EDGE_CURVE('',#42329,#42328,#34266,.T.);
#54515=EDGE_CURVE('',#42330,#42329,#34267,.T.);
#54516=EDGE_CURVE('',#42330,#42325,#22857,.T.);
#54517=EDGE_CURVE('',#42328,#42331,#22858,.T.);
#54518=EDGE_CURVE('',#42331,#42332,#34268,.T.);
#54519=EDGE_CURVE('',#42332,#42329,#22859,.T.);
#54520=EDGE_CURVE('',#40976,#42314,#34269,.T.);
#54521=EDGE_CURVE('',#42313,#40977,#34270,.T.);
#54522=EDGE_CURVE('',#42331,#40473,#1760,.T.);
#54523=EDGE_CURVE('',#40472,#42332,#1761,.T.);
#54524=EDGE_CURVE('',#42323,#42326,#1762,.T.);
#54525=EDGE_CURVE('',#42325,#42324,#1763,.T.);
#54526=EDGE_CURVE('',#42319,#42322,#1764,.T.);
#54527=EDGE_CURVE('',#42321,#42320,#1765,.T.);
#54528=EDGE_CURVE('',#42333,#42334,#34271,.T.);
#54529=EDGE_CURVE('',#42334,#42335,#22860,.T.);
#54530=EDGE_CURVE('',#42336,#42335,#34272,.T.);
#54531=EDGE_CURVE('',#42337,#42336,#34273,.T.);
#54532=EDGE_CURVE('',#42338,#42337,#34274,.T.);
#54533=EDGE_CURVE('',#42338,#42333,#22861,.T.);
#54534=EDGE_CURVE('',#42336,#42339,#22862,.T.);
#54535=EDGE_CURVE('',#42339,#42340,#34275,.T.);
#54536=EDGE_CURVE('',#42340,#42337,#22863,.T.);
#54537=EDGE_CURVE('',#42341,#42342,#34276,.T.);
#54538=EDGE_CURVE('',#42342,#42343,#22864,.T.);
#54539=EDGE_CURVE('',#42343,#42344,#34277,.T.);
#54540=EDGE_CURVE('',#42344,#42341,#22865,.T.);
#54541=EDGE_CURVE('',#42345,#42346,#34278,.T.);
#54542=EDGE_CURVE('',#42346,#42347,#22866,.T.);
#54543=EDGE_CURVE('',#42348,#42347,#34279,.T.);
#54544=EDGE_CURVE('',#42349,#42348,#34280,.T.);
#54545=EDGE_CURVE('',#42350,#42349,#34281,.T.);
#54546=EDGE_CURVE('',#42350,#42345,#22867,.T.);
#54547=EDGE_CURVE('',#42348,#42351,#22868,.T.);
#54548=EDGE_CURVE('',#42351,#42352,#34282,.T.);
#54549=EDGE_CURVE('',#42352,#42349,#22869,.T.);
#54550=EDGE_CURVE('',#40982,#42334,#34283,.T.);
#54551=EDGE_CURVE('',#42333,#40983,#34284,.T.);
#54552=EDGE_CURVE('',#42351,#40467,#1766,.T.);
#54553=EDGE_CURVE('',#40466,#42352,#1767,.T.);
#54554=EDGE_CURVE('',#42343,#42346,#1768,.T.);
#54555=EDGE_CURVE('',#42345,#42344,#1769,.T.);
#54556=EDGE_CURVE('',#42339,#42342,#1770,.T.);
#54557=EDGE_CURVE('',#42341,#42340,#1771,.T.);
#54558=EDGE_CURVE('',#42353,#42354,#34285,.T.);
#54559=EDGE_CURVE('',#42354,#42355,#22870,.T.);
#54560=EDGE_CURVE('',#42356,#42355,#34286,.T.);
#54561=EDGE_CURVE('',#42357,#42356,#34287,.T.);
#54562=EDGE_CURVE('',#42358,#42357,#34288,.T.);
#54563=EDGE_CURVE('',#42358,#42353,#22871,.T.);
#54564=EDGE_CURVE('',#42356,#42359,#22872,.T.);
#54565=EDGE_CURVE('',#42359,#42360,#34289,.T.);
#54566=EDGE_CURVE('',#42360,#42357,#22873,.T.);
#54567=EDGE_CURVE('',#42361,#42362,#34290,.T.);
#54568=EDGE_CURVE('',#42362,#42363,#22874,.T.);
#54569=EDGE_CURVE('',#42363,#42364,#34291,.T.);
#54570=EDGE_CURVE('',#42364,#42361,#22875,.T.);
#54571=EDGE_CURVE('',#42365,#42366,#34292,.T.);
#54572=EDGE_CURVE('',#42366,#42367,#22876,.T.);
#54573=EDGE_CURVE('',#42368,#42367,#34293,.T.);
#54574=EDGE_CURVE('',#42369,#42368,#34294,.T.);
#54575=EDGE_CURVE('',#42370,#42369,#34295,.T.);
#54576=EDGE_CURVE('',#42370,#42365,#22877,.T.);
#54577=EDGE_CURVE('',#42368,#42371,#22878,.T.);
#54578=EDGE_CURVE('',#42371,#42372,#34296,.T.);
#54579=EDGE_CURVE('',#42372,#42369,#22879,.T.);
#54580=EDGE_CURVE('',#40988,#42354,#34297,.T.);
#54581=EDGE_CURVE('',#42353,#40989,#34298,.T.);
#54582=EDGE_CURVE('',#42371,#40461,#1772,.T.);
#54583=EDGE_CURVE('',#40460,#42372,#1773,.T.);
#54584=EDGE_CURVE('',#42363,#42366,#1774,.T.);
#54585=EDGE_CURVE('',#42365,#42364,#1775,.T.);
#54586=EDGE_CURVE('',#42359,#42362,#1776,.T.);
#54587=EDGE_CURVE('',#42361,#42360,#1777,.T.);
#54588=EDGE_CURVE('',#42373,#42374,#22880,.T.);
#54589=EDGE_CURVE('',#42374,#42375,#34299,.T.);
#54590=EDGE_CURVE('',#42375,#42376,#22881,.T.);
#54591=EDGE_CURVE('',#42376,#42373,#34300,.T.);
#54592=EDGE_CURVE('',#42377,#42378,#1778,.T.);
#54593=EDGE_CURVE('',#42378,#42379,#22882,.T.);
#54594=EDGE_CURVE('',#42379,#42380,#22883,.T.);
#54595=EDGE_CURVE('',#42380,#42381,#22884,.T.);
#54596=EDGE_CURVE('',#42381,#42382,#1779,.T.);
#54597=EDGE_CURVE('',#42382,#42383,#22885,.T.);
#54598=EDGE_CURVE('',#42383,#42384,#22886,.T.);
#54599=EDGE_CURVE('',#42384,#42385,#1780,.T.);
#54600=EDGE_CURVE('',#42385,#42386,#22887,.T.);
#54601=EDGE_CURVE('',#42386,#42387,#1781,.T.);
#54602=EDGE_CURVE('',#42387,#42388,#22888,.T.);
#54603=EDGE_CURVE('',#42388,#42377,#22889,.T.);
#54604=EDGE_CURVE('',#42389,#42390,#1782,.T.);
#54605=EDGE_CURVE('',#42390,#42391,#22890,.T.);
#54606=EDGE_CURVE('',#42391,#42392,#22891,.T.);
#54607=EDGE_CURVE('',#42392,#42393,#22892,.T.);
#54608=EDGE_CURVE('',#42393,#42394,#1783,.T.);
#54609=EDGE_CURVE('',#42394,#42395,#22893,.T.);
#54610=EDGE_CURVE('',#42395,#42396,#22894,.T.);
#54611=EDGE_CURVE('',#42396,#42397,#1784,.T.);
#54612=EDGE_CURVE('',#42397,#42398,#22895,.T.);
#54613=EDGE_CURVE('',#42398,#42399,#1785,.T.);
#54614=EDGE_CURVE('',#42399,#42400,#22896,.T.);
#54615=EDGE_CURVE('',#42400,#42389,#22897,.T.);
#54616=EDGE_CURVE('',#42391,#42374,#4975,.T.);
#54617=EDGE_CURVE('',#42373,#42392,#4976,.T.);
#54618=EDGE_CURVE('',#42375,#42380,#4977,.T.);
#54619=EDGE_CURVE('',#42379,#42376,#4978,.T.);
#54620=EDGE_CURVE('',#42400,#42370,#1786,.T.);
#54621=EDGE_CURVE('',#42365,#42399,#34301,.T.);
#54622=EDGE_CURVE('',#42364,#42398,#34302,.T.);
#54623=EDGE_CURVE('',#42389,#42372,#34303,.T.);
#54624=EDGE_CURVE('',#42361,#42397,#34304,.T.);
#54625=EDGE_CURVE('',#42390,#40460,#34305,.T.);
#54626=EDGE_CURVE('',#42360,#42396,#34306,.T.);
#54627=EDGE_CURVE('',#42391,#40459,#34307,.T.);
#54628=EDGE_CURVE('',#42358,#42395,#1787,.T.);
#54629=EDGE_CURVE('',#42374,#40458,#34308,.T.);
#54630=EDGE_CURVE('',#42353,#42394,#34309,.T.);
#54631=EDGE_CURVE('',#42375,#40457,#34310,.T.);
#54632=EDGE_CURVE('',#40989,#42393,#34311,.T.);
#54633=EDGE_CURVE('',#42380,#40812,#34312,.T.);
#54634=EDGE_CURVE('',#40990,#42392,#34313,.T.);
#54635=EDGE_CURVE('',#42381,#40811,#34314,.T.);
#54636=EDGE_CURVE('',#40991,#42373,#34315,.T.);
#54637=EDGE_CURVE('',#42382,#41191,#34316,.T.);
#54638=EDGE_CURVE('',#40993,#42376,#34317,.T.);
#54639=EDGE_CURVE('',#42383,#41189,#1788,.T.);
#54640=EDGE_CURVE('',#40994,#42379,#34318,.T.);
#54641=EDGE_CURVE('',#42384,#41188,#34319,.T.);
#54642=EDGE_CURVE('',#40995,#42378,#34320,.T.);
#54643=EDGE_CURVE('',#42385,#41181,#34321,.T.);
#54644=EDGE_CURVE('',#41176,#42377,#34322,.T.);
#54645=EDGE_CURVE('',#42386,#41184,#34323,.T.);
#54646=EDGE_CURVE('',#41177,#42388,#1789,.T.);
#54647=EDGE_CURVE('',#42387,#41179,#34324,.T.);
#54648=EDGE_CURVE('',#42401,#42402,#22898,.T.);
#54649=EDGE_CURVE('',#42402,#42403,#34325,.T.);
#54650=EDGE_CURVE('',#42403,#42404,#22899,.T.);
#54651=EDGE_CURVE('',#42404,#42401,#34326,.T.);
#54652=EDGE_CURVE('',#42405,#42406,#1790,.T.);
#54653=EDGE_CURVE('',#42406,#42407,#22900,.T.);
#54654=EDGE_CURVE('',#42407,#42408,#22901,.T.);
#54655=EDGE_CURVE('',#42408,#42409,#22902,.T.);
#54656=EDGE_CURVE('',#42409,#42410,#1791,.T.);
#54657=EDGE_CURVE('',#42410,#42411,#22903,.T.);
#54658=EDGE_CURVE('',#42411,#42412,#22904,.T.);
#54659=EDGE_CURVE('',#42412,#42413,#1792,.T.);
#54660=EDGE_CURVE('',#42413,#42414,#22905,.T.);
#54661=EDGE_CURVE('',#42414,#42415,#1793,.T.);
#54662=EDGE_CURVE('',#42415,#42416,#22906,.T.);
#54663=EDGE_CURVE('',#42416,#42405,#22907,.T.);
#54664=EDGE_CURVE('',#42417,#42418,#1794,.T.);
#54665=EDGE_CURVE('',#42418,#42419,#22908,.T.);
#54666=EDGE_CURVE('',#42419,#42420,#22909,.T.);
#54667=EDGE_CURVE('',#42420,#42421,#22910,.T.);
#54668=EDGE_CURVE('',#42421,#42422,#1795,.T.);
#54669=EDGE_CURVE('',#42422,#42423,#22911,.T.);
#54670=EDGE_CURVE('',#42423,#42424,#22912,.T.);
#54671=EDGE_CURVE('',#42424,#42425,#1796,.T.);
#54672=EDGE_CURVE('',#42425,#42426,#22913,.T.);
#54673=EDGE_CURVE('',#42426,#42427,#1797,.T.);
#54674=EDGE_CURVE('',#42427,#42428,#22914,.T.);
#54675=EDGE_CURVE('',#42428,#42417,#22915,.T.);
#54676=EDGE_CURVE('',#42429,#42430,#22916,.T.);
#54677=EDGE_CURVE('',#42430,#42431,#34327,.T.);
#54678=EDGE_CURVE('',#42431,#42432,#22917,.T.);
#54679=EDGE_CURVE('',#42432,#42429,#34328,.T.);
#54680=EDGE_CURVE('',#42433,#42434,#1798,.T.);
#54681=EDGE_CURVE('',#42434,#42435,#22918,.T.);
#54682=EDGE_CURVE('',#42435,#42436,#22919,.T.);
#54683=EDGE_CURVE('',#42436,#42437,#22920,.T.);
#54684=EDGE_CURVE('',#42437,#42438,#1799,.T.);
#54685=EDGE_CURVE('',#42438,#42439,#22921,.T.);
#54686=EDGE_CURVE('',#42439,#42440,#22922,.T.);
#54687=EDGE_CURVE('',#42440,#42441,#1800,.T.);
#54688=EDGE_CURVE('',#42441,#42442,#22923,.T.);
#54689=EDGE_CURVE('',#42442,#42443,#1801,.T.);
#54690=EDGE_CURVE('',#42443,#42444,#22924,.T.);
#54691=EDGE_CURVE('',#42444,#42433,#22925,.T.);
#54692=EDGE_CURVE('',#42445,#42446,#1802,.T.);
#54693=EDGE_CURVE('',#42446,#42447,#22926,.T.);
#54694=EDGE_CURVE('',#42447,#42448,#22927,.T.);
#54695=EDGE_CURVE('',#42448,#42449,#22928,.T.);
#54696=EDGE_CURVE('',#42449,#42450,#1803,.T.);
#54697=EDGE_CURVE('',#42450,#42451,#22929,.T.);
#54698=EDGE_CURVE('',#42451,#42452,#22930,.T.);
#54699=EDGE_CURVE('',#42452,#42453,#1804,.T.);
#54700=EDGE_CURVE('',#42453,#42454,#22931,.T.);
#54701=EDGE_CURVE('',#42454,#42455,#1805,.T.);
#54702=EDGE_CURVE('',#42455,#42456,#22932,.T.);
#54703=EDGE_CURVE('',#42456,#42445,#22933,.T.);
#54704=EDGE_CURVE('',#42457,#42458,#22934,.T.);
#54705=EDGE_CURVE('',#42458,#42459,#34329,.T.);
#54706=EDGE_CURVE('',#42459,#42460,#22935,.T.);
#54707=EDGE_CURVE('',#42460,#42457,#34330,.T.);
#54708=EDGE_CURVE('',#42461,#42462,#1806,.T.);
#54709=EDGE_CURVE('',#42462,#42463,#22936,.T.);
#54710=EDGE_CURVE('',#42463,#42464,#22937,.T.);
#54711=EDGE_CURVE('',#42464,#42465,#22938,.T.);
#54712=EDGE_CURVE('',#42465,#42466,#1807,.T.);
#54713=EDGE_CURVE('',#42466,#42467,#22939,.T.);
#54714=EDGE_CURVE('',#42467,#42468,#22940,.T.);
#54715=EDGE_CURVE('',#42468,#42469,#1808,.T.);
#54716=EDGE_CURVE('',#42469,#42470,#22941,.T.);
#54717=EDGE_CURVE('',#42470,#42471,#1809,.T.);
#54718=EDGE_CURVE('',#42471,#42472,#22942,.T.);
#54719=EDGE_CURVE('',#42472,#42461,#22943,.T.);
#54720=EDGE_CURVE('',#42473,#42474,#1810,.T.);
#54721=EDGE_CURVE('',#42474,#42475,#22944,.T.);
#54722=EDGE_CURVE('',#42475,#42476,#22945,.T.);
#54723=EDGE_CURVE('',#42476,#42477,#22946,.T.);
#54724=EDGE_CURVE('',#42477,#42478,#1811,.T.);
#54725=EDGE_CURVE('',#42478,#42479,#22947,.T.);
#54726=EDGE_CURVE('',#42479,#42480,#22948,.T.);
#54727=EDGE_CURVE('',#42480,#42481,#1812,.T.);
#54728=EDGE_CURVE('',#42481,#42482,#22949,.T.);
#54729=EDGE_CURVE('',#42482,#42483,#1813,.T.);
#54730=EDGE_CURVE('',#42483,#42484,#22950,.T.);
#54731=EDGE_CURVE('',#42484,#42473,#22951,.T.);
#54732=EDGE_CURVE('',#42485,#42486,#22952,.T.);
#54733=EDGE_CURVE('',#42486,#42487,#34331,.T.);
#54734=EDGE_CURVE('',#42487,#42488,#22953,.T.);
#54735=EDGE_CURVE('',#42488,#42485,#34332,.T.);
#54736=EDGE_CURVE('',#42489,#42490,#1814,.T.);
#54737=EDGE_CURVE('',#42490,#42491,#22954,.T.);
#54738=EDGE_CURVE('',#42491,#42492,#22955,.T.);
#54739=EDGE_CURVE('',#42492,#42493,#22956,.T.);
#54740=EDGE_CURVE('',#42493,#42494,#1815,.T.);
#54741=EDGE_CURVE('',#42494,#42495,#22957,.T.);
#54742=EDGE_CURVE('',#42495,#42496,#22958,.T.);
#54743=EDGE_CURVE('',#42496,#42497,#1816,.T.);
#54744=EDGE_CURVE('',#42497,#42498,#22959,.T.);
#54745=EDGE_CURVE('',#42498,#42499,#1817,.T.);
#54746=EDGE_CURVE('',#42499,#42500,#22960,.T.);
#54747=EDGE_CURVE('',#42500,#42489,#22961,.T.);
#54748=EDGE_CURVE('',#42501,#42502,#1818,.T.);
#54749=EDGE_CURVE('',#42502,#42503,#22962,.T.);
#54750=EDGE_CURVE('',#42503,#42504,#22963,.T.);
#54751=EDGE_CURVE('',#42504,#42505,#22964,.T.);
#54752=EDGE_CURVE('',#42505,#42506,#1819,.T.);
#54753=EDGE_CURVE('',#42506,#42507,#22965,.T.);
#54754=EDGE_CURVE('',#42507,#42508,#22966,.T.);
#54755=EDGE_CURVE('',#42508,#42509,#1820,.T.);
#54756=EDGE_CURVE('',#42509,#42510,#22967,.T.);
#54757=EDGE_CURVE('',#42510,#42511,#1821,.T.);
#54758=EDGE_CURVE('',#42511,#42512,#22968,.T.);
#54759=EDGE_CURVE('',#42512,#42501,#22969,.T.);
#54760=EDGE_CURVE('',#42513,#42514,#22970,.T.);
#54761=EDGE_CURVE('',#42514,#42515,#34333,.T.);
#54762=EDGE_CURVE('',#42515,#42516,#22971,.T.);
#54763=EDGE_CURVE('',#42516,#42513,#34334,.T.);
#54764=EDGE_CURVE('',#42517,#42518,#1822,.T.);
#54765=EDGE_CURVE('',#42518,#42519,#22972,.T.);
#54766=EDGE_CURVE('',#42519,#42520,#22973,.T.);
#54767=EDGE_CURVE('',#42520,#42521,#22974,.T.);
#54768=EDGE_CURVE('',#42521,#42522,#1823,.T.);
#54769=EDGE_CURVE('',#42522,#42523,#22975,.T.);
#54770=EDGE_CURVE('',#42523,#42524,#22976,.T.);
#54771=EDGE_CURVE('',#42524,#42525,#1824,.T.);
#54772=EDGE_CURVE('',#42525,#42526,#22977,.T.);
#54773=EDGE_CURVE('',#42526,#42527,#1825,.T.);
#54774=EDGE_CURVE('',#42527,#42528,#22978,.T.);
#54775=EDGE_CURVE('',#42528,#42517,#22979,.T.);
#54776=EDGE_CURVE('',#42529,#42530,#1826,.T.);
#54777=EDGE_CURVE('',#42530,#42531,#22980,.T.);
#54778=EDGE_CURVE('',#42531,#42532,#22981,.T.);
#54779=EDGE_CURVE('',#42532,#42533,#22982,.T.);
#54780=EDGE_CURVE('',#42533,#42534,#1827,.T.);
#54781=EDGE_CURVE('',#42534,#42535,#22983,.T.);
#54782=EDGE_CURVE('',#42535,#42536,#22984,.T.);
#54783=EDGE_CURVE('',#42536,#42537,#1828,.T.);
#54784=EDGE_CURVE('',#42537,#42538,#22985,.T.);
#54785=EDGE_CURVE('',#42538,#42539,#1829,.T.);
#54786=EDGE_CURVE('',#42539,#42540,#22986,.T.);
#54787=EDGE_CURVE('',#42540,#42529,#22987,.T.);
#54788=EDGE_CURVE('',#42541,#42542,#22988,.T.);
#54789=EDGE_CURVE('',#42542,#42543,#34335,.T.);
#54790=EDGE_CURVE('',#42543,#42544,#22989,.T.);
#54791=EDGE_CURVE('',#42544,#42541,#34336,.T.);
#54792=EDGE_CURVE('',#42545,#42546,#1830,.T.);
#54793=EDGE_CURVE('',#42546,#42547,#22990,.T.);
#54794=EDGE_CURVE('',#42547,#42548,#22991,.T.);
#54795=EDGE_CURVE('',#42548,#42549,#22992,.T.);
#54796=EDGE_CURVE('',#42549,#42550,#1831,.T.);
#54797=EDGE_CURVE('',#42550,#42551,#22993,.T.);
#54798=EDGE_CURVE('',#42551,#42552,#22994,.T.);
#54799=EDGE_CURVE('',#42552,#42553,#1832,.T.);
#54800=EDGE_CURVE('',#42553,#42554,#22995,.T.);
#54801=EDGE_CURVE('',#42554,#42555,#1833,.T.);
#54802=EDGE_CURVE('',#42555,#42556,#22996,.T.);
#54803=EDGE_CURVE('',#42556,#42545,#22997,.T.);
#54804=EDGE_CURVE('',#42557,#42558,#1834,.T.);
#54805=EDGE_CURVE('',#42558,#42559,#22998,.T.);
#54806=EDGE_CURVE('',#42559,#42560,#22999,.T.);
#54807=EDGE_CURVE('',#42560,#42561,#23000,.T.);
#54808=EDGE_CURVE('',#42561,#42562,#1835,.T.);
#54809=EDGE_CURVE('',#42562,#42563,#23001,.T.);
#54810=EDGE_CURVE('',#42563,#42564,#23002,.T.);
#54811=EDGE_CURVE('',#42564,#42565,#1836,.T.);
#54812=EDGE_CURVE('',#42565,#42566,#23003,.T.);
#54813=EDGE_CURVE('',#42566,#42567,#1837,.T.);
#54814=EDGE_CURVE('',#42567,#42568,#23004,.T.);
#54815=EDGE_CURVE('',#42568,#42557,#23005,.T.);
#54816=EDGE_CURVE('',#42569,#42570,#23006,.T.);
#54817=EDGE_CURVE('',#42570,#42571,#34337,.T.);
#54818=EDGE_CURVE('',#42571,#42572,#23007,.T.);
#54819=EDGE_CURVE('',#42572,#42569,#34338,.T.);
#54820=EDGE_CURVE('',#42573,#42574,#1838,.T.);
#54821=EDGE_CURVE('',#42574,#42575,#23008,.T.);
#54822=EDGE_CURVE('',#42575,#42576,#23009,.T.);
#54823=EDGE_CURVE('',#42576,#42577,#23010,.T.);
#54824=EDGE_CURVE('',#42577,#42578,#1839,.T.);
#54825=EDGE_CURVE('',#42578,#42579,#23011,.T.);
#54826=EDGE_CURVE('',#42579,#42580,#23012,.T.);
#54827=EDGE_CURVE('',#42580,#42581,#1840,.T.);
#54828=EDGE_CURVE('',#42581,#42582,#23013,.T.);
#54829=EDGE_CURVE('',#42582,#42583,#1841,.T.);
#54830=EDGE_CURVE('',#42583,#42584,#23014,.T.);
#54831=EDGE_CURVE('',#42584,#42573,#23015,.T.);
#54832=EDGE_CURVE('',#42585,#42586,#1842,.T.);
#54833=EDGE_CURVE('',#42586,#42587,#23016,.T.);
#54834=EDGE_CURVE('',#42587,#42588,#23017,.T.);
#54835=EDGE_CURVE('',#42588,#42589,#23018,.T.);
#54836=EDGE_CURVE('',#42589,#42590,#1843,.T.);
#54837=EDGE_CURVE('',#42590,#42591,#23019,.T.);
#54838=EDGE_CURVE('',#42591,#42592,#23020,.T.);
#54839=EDGE_CURVE('',#42592,#42593,#1844,.T.);
#54840=EDGE_CURVE('',#42593,#42594,#23021,.T.);
#54841=EDGE_CURVE('',#42594,#42595,#1845,.T.);
#54842=EDGE_CURVE('',#42595,#42596,#23022,.T.);
#54843=EDGE_CURVE('',#42596,#42585,#23023,.T.);
#54844=EDGE_CURVE('',#42597,#42598,#23024,.T.);
#54845=EDGE_CURVE('',#42598,#42599,#34339,.T.);
#54846=EDGE_CURVE('',#42599,#42600,#23025,.T.);
#54847=EDGE_CURVE('',#42600,#42597,#34340,.T.);
#54848=EDGE_CURVE('',#42601,#42602,#1846,.T.);
#54849=EDGE_CURVE('',#42602,#42603,#23026,.T.);
#54850=EDGE_CURVE('',#42603,#42604,#23027,.T.);
#54851=EDGE_CURVE('',#42604,#42605,#23028,.T.);
#54852=EDGE_CURVE('',#42605,#42606,#1847,.T.);
#54853=EDGE_CURVE('',#42606,#42607,#23029,.T.);
#54854=EDGE_CURVE('',#42607,#42608,#23030,.T.);
#54855=EDGE_CURVE('',#42608,#42609,#1848,.T.);
#54856=EDGE_CURVE('',#42609,#42610,#23031,.T.);
#54857=EDGE_CURVE('',#42610,#42611,#1849,.T.);
#54858=EDGE_CURVE('',#42611,#42612,#23032,.T.);
#54859=EDGE_CURVE('',#42612,#42601,#23033,.T.);
#54860=EDGE_CURVE('',#42613,#42614,#1850,.T.);
#54861=EDGE_CURVE('',#42614,#42615,#23034,.T.);
#54862=EDGE_CURVE('',#42615,#42616,#23035,.T.);
#54863=EDGE_CURVE('',#42616,#42617,#23036,.T.);
#54864=EDGE_CURVE('',#42617,#42618,#1851,.T.);
#54865=EDGE_CURVE('',#42618,#42619,#23037,.T.);
#54866=EDGE_CURVE('',#42619,#42620,#23038,.T.);
#54867=EDGE_CURVE('',#42620,#42621,#1852,.T.);
#54868=EDGE_CURVE('',#42621,#42622,#23039,.T.);
#54869=EDGE_CURVE('',#42622,#42623,#1853,.T.);
#54870=EDGE_CURVE('',#42623,#42624,#23040,.T.);
#54871=EDGE_CURVE('',#42624,#42613,#23041,.T.);
#54872=EDGE_CURVE('',#42625,#42626,#23042,.T.);
#54873=EDGE_CURVE('',#42626,#42627,#34341,.T.);
#54874=EDGE_CURVE('',#42627,#42628,#23043,.T.);
#54875=EDGE_CURVE('',#42628,#42625,#34342,.T.);
#54876=EDGE_CURVE('',#42629,#42630,#1854,.T.);
#54877=EDGE_CURVE('',#42630,#42631,#23044,.T.);
#54878=EDGE_CURVE('',#42631,#42632,#23045,.T.);
#54879=EDGE_CURVE('',#42632,#42633,#23046,.T.);
#54880=EDGE_CURVE('',#42633,#42634,#1855,.T.);
#54881=EDGE_CURVE('',#42634,#42635,#23047,.T.);
#54882=EDGE_CURVE('',#42635,#42636,#23048,.T.);
#54883=EDGE_CURVE('',#42636,#42637,#1856,.T.);
#54884=EDGE_CURVE('',#42637,#42638,#23049,.T.);
#54885=EDGE_CURVE('',#42638,#42639,#1857,.T.);
#54886=EDGE_CURVE('',#42639,#42640,#23050,.T.);
#54887=EDGE_CURVE('',#42640,#42629,#23051,.T.);
#54888=EDGE_CURVE('',#42641,#42642,#1858,.T.);
#54889=EDGE_CURVE('',#42642,#42643,#23052,.T.);
#54890=EDGE_CURVE('',#42643,#42644,#23053,.T.);
#54891=EDGE_CURVE('',#42644,#42645,#23054,.T.);
#54892=EDGE_CURVE('',#42645,#42646,#1859,.T.);
#54893=EDGE_CURVE('',#42646,#42647,#23055,.T.);
#54894=EDGE_CURVE('',#42647,#42648,#23056,.T.);
#54895=EDGE_CURVE('',#42648,#42649,#1860,.T.);
#54896=EDGE_CURVE('',#42649,#42650,#23057,.T.);
#54897=EDGE_CURVE('',#42650,#42651,#1861,.T.);
#54898=EDGE_CURVE('',#42651,#42652,#23058,.T.);
#54899=EDGE_CURVE('',#42652,#42641,#23059,.T.);
#54900=EDGE_CURVE('',#42653,#42654,#23060,.T.);
#54901=EDGE_CURVE('',#42654,#42655,#34343,.T.);
#54902=EDGE_CURVE('',#42655,#42656,#23061,.T.);
#54903=EDGE_CURVE('',#42656,#42653,#34344,.T.);
#54904=EDGE_CURVE('',#42657,#42658,#1862,.T.);
#54905=EDGE_CURVE('',#42658,#42659,#23062,.T.);
#54906=EDGE_CURVE('',#42659,#42660,#23063,.T.);
#54907=EDGE_CURVE('',#42660,#42661,#23064,.T.);
#54908=EDGE_CURVE('',#42661,#42662,#1863,.T.);
#54909=EDGE_CURVE('',#42662,#42663,#23065,.T.);
#54910=EDGE_CURVE('',#42663,#42664,#23066,.T.);
#54911=EDGE_CURVE('',#42664,#42665,#1864,.T.);
#54912=EDGE_CURVE('',#42665,#42666,#23067,.T.);
#54913=EDGE_CURVE('',#42666,#42667,#1865,.T.);
#54914=EDGE_CURVE('',#42667,#42668,#23068,.T.);
#54915=EDGE_CURVE('',#42668,#42657,#23069,.T.);
#54916=EDGE_CURVE('',#42669,#42670,#1866,.T.);
#54917=EDGE_CURVE('',#42670,#42671,#23070,.T.);
#54918=EDGE_CURVE('',#42671,#42672,#23071,.T.);
#54919=EDGE_CURVE('',#42672,#42673,#23072,.T.);
#54920=EDGE_CURVE('',#42673,#42674,#1867,.T.);
#54921=EDGE_CURVE('',#42674,#42675,#23073,.T.);
#54922=EDGE_CURVE('',#42675,#42676,#23074,.T.);
#54923=EDGE_CURVE('',#42676,#42677,#1868,.T.);
#54924=EDGE_CURVE('',#42677,#42678,#23075,.T.);
#54925=EDGE_CURVE('',#42678,#42679,#1869,.T.);
#54926=EDGE_CURVE('',#42679,#42680,#23076,.T.);
#54927=EDGE_CURVE('',#42680,#42669,#23077,.T.);
#54928=EDGE_CURVE('',#42681,#42682,#23078,.T.);
#54929=EDGE_CURVE('',#42682,#42683,#34345,.T.);
#54930=EDGE_CURVE('',#42683,#42684,#23079,.T.);
#54931=EDGE_CURVE('',#42684,#42681,#34346,.T.);
#54932=EDGE_CURVE('',#42685,#42686,#1870,.T.);
#54933=EDGE_CURVE('',#42686,#42687,#23080,.T.);
#54934=EDGE_CURVE('',#42687,#42688,#23081,.T.);
#54935=EDGE_CURVE('',#42688,#42689,#23082,.T.);
#54936=EDGE_CURVE('',#42689,#42690,#1871,.T.);
#54937=EDGE_CURVE('',#42690,#42691,#23083,.T.);
#54938=EDGE_CURVE('',#42691,#42692,#23084,.T.);
#54939=EDGE_CURVE('',#42692,#42693,#1872,.T.);
#54940=EDGE_CURVE('',#42693,#42694,#23085,.T.);
#54941=EDGE_CURVE('',#42694,#42695,#1873,.T.);
#54942=EDGE_CURVE('',#42695,#42696,#23086,.T.);
#54943=EDGE_CURVE('',#42696,#42685,#23087,.T.);
#54944=EDGE_CURVE('',#42697,#42698,#1874,.T.);
#54945=EDGE_CURVE('',#42698,#42699,#23088,.T.);
#54946=EDGE_CURVE('',#42699,#42700,#23089,.T.);
#54947=EDGE_CURVE('',#42700,#42701,#23090,.T.);
#54948=EDGE_CURVE('',#42701,#42702,#1875,.T.);
#54949=EDGE_CURVE('',#42702,#42703,#23091,.T.);
#54950=EDGE_CURVE('',#42703,#42704,#23092,.T.);
#54951=EDGE_CURVE('',#42704,#42705,#1876,.T.);
#54952=EDGE_CURVE('',#42705,#42706,#23093,.T.);
#54953=EDGE_CURVE('',#42706,#42707,#1877,.T.);
#54954=EDGE_CURVE('',#42707,#42708,#23094,.T.);
#54955=EDGE_CURVE('',#42708,#42697,#23095,.T.);
#54956=EDGE_CURVE('',#42709,#42710,#23096,.T.);
#54957=EDGE_CURVE('',#42710,#42711,#34347,.T.);
#54958=EDGE_CURVE('',#42711,#42712,#23097,.T.);
#54959=EDGE_CURVE('',#42712,#42709,#34348,.T.);
#54960=EDGE_CURVE('',#42713,#42714,#1878,.T.);
#54961=EDGE_CURVE('',#42714,#42715,#23098,.T.);
#54962=EDGE_CURVE('',#42715,#42716,#23099,.T.);
#54963=EDGE_CURVE('',#42716,#42717,#23100,.T.);
#54964=EDGE_CURVE('',#42717,#42718,#1879,.T.);
#54965=EDGE_CURVE('',#42718,#42719,#23101,.T.);
#54966=EDGE_CURVE('',#42719,#42720,#23102,.T.);
#54967=EDGE_CURVE('',#42720,#42721,#1880,.T.);
#54968=EDGE_CURVE('',#42721,#42722,#23103,.T.);
#54969=EDGE_CURVE('',#42722,#42723,#1881,.T.);
#54970=EDGE_CURVE('',#42723,#42724,#23104,.T.);
#54971=EDGE_CURVE('',#42724,#42713,#23105,.T.);
#54972=EDGE_CURVE('',#42725,#42726,#1882,.T.);
#54973=EDGE_CURVE('',#42726,#42727,#23106,.T.);
#54974=EDGE_CURVE('',#42727,#42728,#23107,.T.);
#54975=EDGE_CURVE('',#42728,#42729,#23108,.T.);
#54976=EDGE_CURVE('',#42729,#42730,#1883,.T.);
#54977=EDGE_CURVE('',#42730,#42731,#23109,.T.);
#54978=EDGE_CURVE('',#42731,#42732,#23110,.T.);
#54979=EDGE_CURVE('',#42732,#42733,#1884,.T.);
#54980=EDGE_CURVE('',#42733,#42734,#23111,.T.);
#54981=EDGE_CURVE('',#42734,#42735,#1885,.T.);
#54982=EDGE_CURVE('',#42735,#42736,#23112,.T.);
#54983=EDGE_CURVE('',#42736,#42725,#23113,.T.);
#54984=EDGE_CURVE('',#42737,#42738,#23114,.T.);
#54985=EDGE_CURVE('',#42738,#42739,#34349,.T.);
#54986=EDGE_CURVE('',#42739,#42740,#23115,.T.);
#54987=EDGE_CURVE('',#42740,#42737,#34350,.T.);
#54988=EDGE_CURVE('',#42741,#42742,#1886,.T.);
#54989=EDGE_CURVE('',#42742,#42743,#23116,.T.);
#54990=EDGE_CURVE('',#42743,#42744,#23117,.T.);
#54991=EDGE_CURVE('',#42744,#42745,#23118,.T.);
#54992=EDGE_CURVE('',#42745,#42746,#1887,.T.);
#54993=EDGE_CURVE('',#42746,#42747,#23119,.T.);
#54994=EDGE_CURVE('',#42747,#42748,#23120,.T.);
#54995=EDGE_CURVE('',#42748,#42749,#1888,.T.);
#54996=EDGE_CURVE('',#42749,#42750,#23121,.T.);
#54997=EDGE_CURVE('',#42750,#42751,#1889,.T.);
#54998=EDGE_CURVE('',#42751,#42752,#23122,.T.);
#54999=EDGE_CURVE('',#42752,#42741,#23123,.T.);
#55000=EDGE_CURVE('',#42753,#42754,#1890,.T.);
#55001=EDGE_CURVE('',#42754,#42755,#23124,.T.);
#55002=EDGE_CURVE('',#42755,#42756,#23125,.T.);
#55003=EDGE_CURVE('',#42756,#42757,#23126,.T.);
#55004=EDGE_CURVE('',#42757,#42758,#1891,.T.);
#55005=EDGE_CURVE('',#42758,#42759,#23127,.T.);
#55006=EDGE_CURVE('',#42759,#42760,#23128,.T.);
#55007=EDGE_CURVE('',#42760,#42761,#1892,.T.);
#55008=EDGE_CURVE('',#42761,#42762,#23129,.T.);
#55009=EDGE_CURVE('',#42762,#42763,#1893,.T.);
#55010=EDGE_CURVE('',#42763,#42764,#23130,.T.);
#55011=EDGE_CURVE('',#42764,#42753,#23131,.T.);
#55012=EDGE_CURVE('',#42765,#42766,#23132,.T.);
#55013=EDGE_CURVE('',#42766,#42767,#34351,.T.);
#55014=EDGE_CURVE('',#42767,#42768,#23133,.T.);
#55015=EDGE_CURVE('',#42768,#42765,#34352,.T.);
#55016=EDGE_CURVE('',#42769,#42770,#1894,.T.);
#55017=EDGE_CURVE('',#42770,#42771,#23134,.T.);
#55018=EDGE_CURVE('',#42771,#42772,#23135,.T.);
#55019=EDGE_CURVE('',#42772,#42773,#23136,.T.);
#55020=EDGE_CURVE('',#42773,#42774,#1895,.T.);
#55021=EDGE_CURVE('',#42774,#42775,#23137,.T.);
#55022=EDGE_CURVE('',#42775,#42776,#23138,.T.);
#55023=EDGE_CURVE('',#42776,#42777,#1896,.T.);
#55024=EDGE_CURVE('',#42777,#42778,#23139,.T.);
#55025=EDGE_CURVE('',#42778,#42779,#1897,.T.);
#55026=EDGE_CURVE('',#42779,#42780,#23140,.T.);
#55027=EDGE_CURVE('',#42780,#42769,#23141,.T.);
#55028=EDGE_CURVE('',#42781,#42782,#1898,.T.);
#55029=EDGE_CURVE('',#42782,#42783,#23142,.T.);
#55030=EDGE_CURVE('',#42783,#42784,#23143,.T.);
#55031=EDGE_CURVE('',#42784,#42785,#23144,.T.);
#55032=EDGE_CURVE('',#42785,#42786,#1899,.T.);
#55033=EDGE_CURVE('',#42786,#42787,#23145,.T.);
#55034=EDGE_CURVE('',#42787,#42788,#23146,.T.);
#55035=EDGE_CURVE('',#42788,#42789,#1900,.T.);
#55036=EDGE_CURVE('',#42789,#42790,#23147,.T.);
#55037=EDGE_CURVE('',#42790,#42791,#1901,.T.);
#55038=EDGE_CURVE('',#42791,#42792,#23148,.T.);
#55039=EDGE_CURVE('',#42792,#42781,#23149,.T.);
#55040=EDGE_CURVE('',#42793,#42794,#23150,.T.);
#55041=EDGE_CURVE('',#42794,#42795,#34353,.T.);
#55042=EDGE_CURVE('',#42795,#42796,#23151,.T.);
#55043=EDGE_CURVE('',#42796,#42793,#34354,.T.);
#55044=EDGE_CURVE('',#42797,#42798,#1902,.T.);
#55045=EDGE_CURVE('',#42798,#42799,#23152,.T.);
#55046=EDGE_CURVE('',#42799,#42800,#23153,.T.);
#55047=EDGE_CURVE('',#42800,#42801,#23154,.T.);
#55048=EDGE_CURVE('',#42801,#42802,#1903,.T.);
#55049=EDGE_CURVE('',#42802,#42803,#23155,.T.);
#55050=EDGE_CURVE('',#42803,#42804,#23156,.T.);
#55051=EDGE_CURVE('',#42804,#42805,#1904,.T.);
#55052=EDGE_CURVE('',#42805,#42806,#23157,.T.);
#55053=EDGE_CURVE('',#42806,#42807,#1905,.T.);
#55054=EDGE_CURVE('',#42807,#42808,#23158,.T.);
#55055=EDGE_CURVE('',#42808,#42797,#23159,.T.);
#55056=EDGE_CURVE('',#42809,#42810,#1906,.T.);
#55057=EDGE_CURVE('',#42810,#42811,#23160,.T.);
#55058=EDGE_CURVE('',#42811,#42812,#23161,.T.);
#55059=EDGE_CURVE('',#42812,#42813,#23162,.T.);
#55060=EDGE_CURVE('',#42813,#42814,#1907,.T.);
#55061=EDGE_CURVE('',#42814,#42815,#23163,.T.);
#55062=EDGE_CURVE('',#42815,#42816,#23164,.T.);
#55063=EDGE_CURVE('',#42816,#42817,#1908,.T.);
#55064=EDGE_CURVE('',#42817,#42818,#23165,.T.);
#55065=EDGE_CURVE('',#42818,#42819,#1909,.T.);
#55066=EDGE_CURVE('',#42819,#42820,#23166,.T.);
#55067=EDGE_CURVE('',#42820,#42809,#23167,.T.);
#55068=EDGE_CURVE('',#42821,#42822,#23168,.T.);
#55069=EDGE_CURVE('',#42822,#42823,#34355,.T.);
#55070=EDGE_CURVE('',#42823,#42824,#23169,.T.);
#55071=EDGE_CURVE('',#42824,#42821,#34356,.T.);
#55072=EDGE_CURVE('',#42825,#42826,#1910,.T.);
#55073=EDGE_CURVE('',#42826,#42827,#23170,.T.);
#55074=EDGE_CURVE('',#42827,#42828,#23171,.T.);
#55075=EDGE_CURVE('',#42828,#42829,#23172,.T.);
#55076=EDGE_CURVE('',#42829,#42830,#1911,.T.);
#55077=EDGE_CURVE('',#42830,#42831,#23173,.T.);
#55078=EDGE_CURVE('',#42831,#42832,#23174,.T.);
#55079=EDGE_CURVE('',#42832,#42833,#1912,.T.);
#55080=EDGE_CURVE('',#42833,#42834,#23175,.T.);
#55081=EDGE_CURVE('',#42834,#42835,#1913,.T.);
#55082=EDGE_CURVE('',#42835,#42836,#23176,.T.);
#55083=EDGE_CURVE('',#42836,#42825,#23177,.T.);
#55084=EDGE_CURVE('',#42837,#42838,#1914,.T.);
#55085=EDGE_CURVE('',#42838,#42839,#23178,.T.);
#55086=EDGE_CURVE('',#42839,#42840,#23179,.T.);
#55087=EDGE_CURVE('',#42840,#42841,#23180,.T.);
#55088=EDGE_CURVE('',#42841,#42842,#1915,.T.);
#55089=EDGE_CURVE('',#42842,#42843,#23181,.T.);
#55090=EDGE_CURVE('',#42843,#42844,#23182,.T.);
#55091=EDGE_CURVE('',#42844,#42845,#1916,.T.);
#55092=EDGE_CURVE('',#42845,#42846,#23183,.T.);
#55093=EDGE_CURVE('',#42846,#42847,#1917,.T.);
#55094=EDGE_CURVE('',#42847,#42848,#23184,.T.);
#55095=EDGE_CURVE('',#42848,#42837,#23185,.T.);
#55096=EDGE_CURVE('',#42849,#42850,#23186,.T.);
#55097=EDGE_CURVE('',#42850,#42851,#34357,.T.);
#55098=EDGE_CURVE('',#42851,#42852,#23187,.T.);
#55099=EDGE_CURVE('',#42852,#42849,#34358,.T.);
#55100=EDGE_CURVE('',#42853,#42854,#1918,.T.);
#55101=EDGE_CURVE('',#42854,#42855,#23188,.T.);
#55102=EDGE_CURVE('',#42855,#42856,#23189,.T.);
#55103=EDGE_CURVE('',#42856,#42857,#23190,.T.);
#55104=EDGE_CURVE('',#42857,#42858,#1919,.T.);
#55105=EDGE_CURVE('',#42858,#42859,#23191,.T.);
#55106=EDGE_CURVE('',#42859,#42860,#23192,.T.);
#55107=EDGE_CURVE('',#42860,#42861,#1920,.T.);
#55108=EDGE_CURVE('',#42861,#42862,#23193,.T.);
#55109=EDGE_CURVE('',#42862,#42863,#1921,.T.);
#55110=EDGE_CURVE('',#42863,#42864,#23194,.T.);
#55111=EDGE_CURVE('',#42864,#42853,#23195,.T.);
#55112=EDGE_CURVE('',#42865,#42866,#1922,.T.);
#55113=EDGE_CURVE('',#42866,#42867,#23196,.T.);
#55114=EDGE_CURVE('',#42867,#42868,#23197,.T.);
#55115=EDGE_CURVE('',#42868,#42869,#23198,.T.);
#55116=EDGE_CURVE('',#42869,#42870,#1923,.T.);
#55117=EDGE_CURVE('',#42870,#42871,#23199,.T.);
#55118=EDGE_CURVE('',#42871,#42872,#23200,.T.);
#55119=EDGE_CURVE('',#42872,#42873,#1924,.T.);
#55120=EDGE_CURVE('',#42873,#42874,#23201,.T.);
#55121=EDGE_CURVE('',#42874,#42875,#1925,.T.);
#55122=EDGE_CURVE('',#42875,#42876,#23202,.T.);
#55123=EDGE_CURVE('',#42876,#42865,#23203,.T.);
#55124=EDGE_CURVE('',#42877,#42878,#23204,.T.);
#55125=EDGE_CURVE('',#42878,#42879,#34359,.T.);
#55126=EDGE_CURVE('',#42879,#42880,#23205,.T.);
#55127=EDGE_CURVE('',#42880,#42877,#34360,.T.);
#55128=EDGE_CURVE('',#42881,#42882,#1926,.T.);
#55129=EDGE_CURVE('',#42882,#42883,#23206,.T.);
#55130=EDGE_CURVE('',#42883,#42884,#23207,.T.);
#55131=EDGE_CURVE('',#42884,#42885,#23208,.T.);
#55132=EDGE_CURVE('',#42885,#42886,#1927,.T.);
#55133=EDGE_CURVE('',#42886,#42887,#23209,.T.);
#55134=EDGE_CURVE('',#42887,#42888,#23210,.T.);
#55135=EDGE_CURVE('',#42888,#42889,#1928,.T.);
#55136=EDGE_CURVE('',#42889,#42890,#23211,.T.);
#55137=EDGE_CURVE('',#42890,#42891,#1929,.T.);
#55138=EDGE_CURVE('',#42891,#42892,#23212,.T.);
#55139=EDGE_CURVE('',#42892,#42881,#23213,.T.);
#55140=EDGE_CURVE('',#42893,#42894,#1930,.T.);
#55141=EDGE_CURVE('',#42894,#42895,#23214,.T.);
#55142=EDGE_CURVE('',#42895,#42896,#23215,.T.);
#55143=EDGE_CURVE('',#42896,#42897,#23216,.T.);
#55144=EDGE_CURVE('',#42897,#42898,#1931,.T.);
#55145=EDGE_CURVE('',#42898,#42899,#23217,.T.);
#55146=EDGE_CURVE('',#42899,#42900,#23218,.T.);
#55147=EDGE_CURVE('',#42900,#42901,#1932,.T.);
#55148=EDGE_CURVE('',#42901,#42902,#23219,.T.);
#55149=EDGE_CURVE('',#42902,#42903,#1933,.T.);
#55150=EDGE_CURVE('',#42903,#42904,#23220,.T.);
#55151=EDGE_CURVE('',#42904,#42893,#23221,.T.);
#55152=EDGE_CURVE('',#42905,#42906,#23222,.T.);
#55153=EDGE_CURVE('',#42906,#42907,#34361,.T.);
#55154=EDGE_CURVE('',#42907,#42908,#23223,.T.);
#55155=EDGE_CURVE('',#42908,#42905,#34362,.T.);
#55156=EDGE_CURVE('',#42909,#42910,#1934,.T.);
#55157=EDGE_CURVE('',#42910,#42911,#23224,.T.);
#55158=EDGE_CURVE('',#42911,#42912,#23225,.T.);
#55159=EDGE_CURVE('',#42912,#42913,#23226,.T.);
#55160=EDGE_CURVE('',#42913,#42914,#1935,.T.);
#55161=EDGE_CURVE('',#42914,#42915,#23227,.T.);
#55162=EDGE_CURVE('',#42915,#42916,#23228,.T.);
#55163=EDGE_CURVE('',#42916,#42917,#1936,.T.);
#55164=EDGE_CURVE('',#42917,#42918,#23229,.T.);
#55165=EDGE_CURVE('',#42918,#42919,#1937,.T.);
#55166=EDGE_CURVE('',#42919,#42920,#23230,.T.);
#55167=EDGE_CURVE('',#42920,#42909,#23231,.T.);
#55168=EDGE_CURVE('',#42921,#42922,#1938,.T.);
#55169=EDGE_CURVE('',#42922,#42923,#23232,.T.);
#55170=EDGE_CURVE('',#42923,#42924,#23233,.T.);
#55171=EDGE_CURVE('',#42924,#42925,#23234,.T.);
#55172=EDGE_CURVE('',#42925,#42926,#1939,.T.);
#55173=EDGE_CURVE('',#42926,#42927,#23235,.T.);
#55174=EDGE_CURVE('',#42927,#42928,#23236,.T.);
#55175=EDGE_CURVE('',#42928,#42929,#1940,.T.);
#55176=EDGE_CURVE('',#42929,#42930,#23237,.T.);
#55177=EDGE_CURVE('',#42930,#42931,#1941,.T.);
#55178=EDGE_CURVE('',#42931,#42932,#23238,.T.);
#55179=EDGE_CURVE('',#42932,#42921,#23239,.T.);
#55180=EDGE_CURVE('',#42933,#42934,#23240,.T.);
#55181=EDGE_CURVE('',#42934,#42935,#34363,.T.);
#55182=EDGE_CURVE('',#42935,#42936,#23241,.T.);
#55183=EDGE_CURVE('',#42936,#42933,#34364,.T.);
#55184=EDGE_CURVE('',#42937,#42938,#1942,.T.);
#55185=EDGE_CURVE('',#42938,#42939,#23242,.T.);
#55186=EDGE_CURVE('',#42939,#42940,#23243,.T.);
#55187=EDGE_CURVE('',#42940,#42941,#23244,.T.);
#55188=EDGE_CURVE('',#42941,#42942,#1943,.T.);
#55189=EDGE_CURVE('',#42942,#42943,#23245,.T.);
#55190=EDGE_CURVE('',#42943,#42944,#23246,.T.);
#55191=EDGE_CURVE('',#42944,#42945,#1944,.T.);
#55192=EDGE_CURVE('',#42945,#42946,#23247,.T.);
#55193=EDGE_CURVE('',#42946,#42947,#1945,.T.);
#55194=EDGE_CURVE('',#42947,#42948,#23248,.T.);
#55195=EDGE_CURVE('',#42948,#42937,#23249,.T.);
#55196=EDGE_CURVE('',#42949,#42950,#1946,.T.);
#55197=EDGE_CURVE('',#42950,#42951,#23250,.T.);
#55198=EDGE_CURVE('',#42951,#42952,#23251,.T.);
#55199=EDGE_CURVE('',#42952,#42953,#23252,.T.);
#55200=EDGE_CURVE('',#42953,#42954,#1947,.T.);
#55201=EDGE_CURVE('',#42954,#42955,#23253,.T.);
#55202=EDGE_CURVE('',#42955,#42956,#23254,.T.);
#55203=EDGE_CURVE('',#42956,#42957,#1948,.T.);
#55204=EDGE_CURVE('',#42957,#42958,#23255,.T.);
#55205=EDGE_CURVE('',#42958,#42959,#1949,.T.);
#55206=EDGE_CURVE('',#42959,#42960,#23256,.T.);
#55207=EDGE_CURVE('',#42960,#42949,#23257,.T.);
#55208=EDGE_CURVE('',#42961,#42962,#23258,.T.);
#55209=EDGE_CURVE('',#42962,#42963,#34365,.T.);
#55210=EDGE_CURVE('',#42963,#42964,#23259,.T.);
#55211=EDGE_CURVE('',#42964,#42961,#34366,.T.);
#55212=EDGE_CURVE('',#42965,#42966,#1950,.T.);
#55213=EDGE_CURVE('',#42966,#42967,#23260,.T.);
#55214=EDGE_CURVE('',#42967,#42968,#23261,.T.);
#55215=EDGE_CURVE('',#42968,#42969,#23262,.T.);
#55216=EDGE_CURVE('',#42969,#42970,#1951,.T.);
#55217=EDGE_CURVE('',#42970,#42971,#23263,.T.);
#55218=EDGE_CURVE('',#42971,#42972,#23264,.T.);
#55219=EDGE_CURVE('',#42972,#42973,#1952,.T.);
#55220=EDGE_CURVE('',#42973,#42974,#23265,.T.);
#55221=EDGE_CURVE('',#42974,#42975,#1953,.T.);
#55222=EDGE_CURVE('',#42975,#42976,#23266,.T.);
#55223=EDGE_CURVE('',#42976,#42965,#23267,.T.);
#55224=EDGE_CURVE('',#42977,#42978,#1954,.T.);
#55225=EDGE_CURVE('',#42978,#42979,#23268,.T.);
#55226=EDGE_CURVE('',#42979,#42980,#23269,.T.);
#55227=EDGE_CURVE('',#42980,#42981,#23270,.T.);
#55228=EDGE_CURVE('',#42981,#42982,#1955,.T.);
#55229=EDGE_CURVE('',#42982,#42983,#23271,.T.);
#55230=EDGE_CURVE('',#42983,#42984,#23272,.T.);
#55231=EDGE_CURVE('',#42984,#42985,#1956,.T.);
#55232=EDGE_CURVE('',#42985,#42986,#23273,.T.);
#55233=EDGE_CURVE('',#42986,#42987,#1957,.T.);
#55234=EDGE_CURVE('',#42987,#42988,#23274,.T.);
#55235=EDGE_CURVE('',#42988,#42977,#23275,.T.);
#55236=EDGE_CURVE('',#42989,#42990,#23276,.T.);
#55237=EDGE_CURVE('',#42990,#42991,#34367,.T.);
#55238=EDGE_CURVE('',#42991,#42992,#23277,.T.);
#55239=EDGE_CURVE('',#42992,#42989,#34368,.T.);
#55240=EDGE_CURVE('',#42993,#42994,#1958,.T.);
#55241=EDGE_CURVE('',#42994,#42995,#23278,.T.);
#55242=EDGE_CURVE('',#42995,#42996,#23279,.T.);
#55243=EDGE_CURVE('',#42996,#42997,#23280,.T.);
#55244=EDGE_CURVE('',#42997,#42998,#1959,.T.);
#55245=EDGE_CURVE('',#42998,#42999,#23281,.T.);
#55246=EDGE_CURVE('',#42999,#43000,#23282,.T.);
#55247=EDGE_CURVE('',#43000,#43001,#1960,.T.);
#55248=EDGE_CURVE('',#43001,#43002,#23283,.T.);
#55249=EDGE_CURVE('',#43002,#43003,#1961,.T.);
#55250=EDGE_CURVE('',#43003,#43004,#23284,.T.);
#55251=EDGE_CURVE('',#43004,#42993,#23285,.T.);
#55252=EDGE_CURVE('',#43005,#43006,#1962,.T.);
#55253=EDGE_CURVE('',#43006,#43007,#23286,.T.);
#55254=EDGE_CURVE('',#43007,#43008,#23287,.T.);
#55255=EDGE_CURVE('',#43008,#43009,#23288,.T.);
#55256=EDGE_CURVE('',#43009,#43010,#1963,.T.);
#55257=EDGE_CURVE('',#43010,#43011,#23289,.T.);
#55258=EDGE_CURVE('',#43011,#43012,#23290,.T.);
#55259=EDGE_CURVE('',#43012,#43013,#1964,.T.);
#55260=EDGE_CURVE('',#43013,#43014,#23291,.T.);
#55261=EDGE_CURVE('',#43014,#43015,#1965,.T.);
#55262=EDGE_CURVE('',#43015,#43016,#23292,.T.);
#55263=EDGE_CURVE('',#43016,#43005,#23293,.T.);
#55264=EDGE_CURVE('',#43017,#43018,#23294,.T.);
#55265=EDGE_CURVE('',#43018,#43019,#34369,.T.);
#55266=EDGE_CURVE('',#43019,#43020,#23295,.T.);
#55267=EDGE_CURVE('',#43020,#43017,#34370,.T.);
#55268=EDGE_CURVE('',#43021,#43022,#1966,.T.);
#55269=EDGE_CURVE('',#43022,#43023,#23296,.T.);
#55270=EDGE_CURVE('',#43023,#43024,#23297,.T.);
#55271=EDGE_CURVE('',#43024,#43025,#23298,.T.);
#55272=EDGE_CURVE('',#43025,#43026,#1967,.T.);
#55273=EDGE_CURVE('',#43026,#43027,#23299,.T.);
#55274=EDGE_CURVE('',#43027,#43028,#23300,.T.);
#55275=EDGE_CURVE('',#43028,#43029,#1968,.T.);
#55276=EDGE_CURVE('',#43029,#43030,#23301,.T.);
#55277=EDGE_CURVE('',#43030,#43031,#1969,.T.);
#55278=EDGE_CURVE('',#43031,#43032,#23302,.T.);
#55279=EDGE_CURVE('',#43032,#43021,#23303,.T.);
#55280=EDGE_CURVE('',#43033,#43034,#1970,.T.);
#55281=EDGE_CURVE('',#43034,#43035,#23304,.T.);
#55282=EDGE_CURVE('',#43035,#43036,#23305,.T.);
#55283=EDGE_CURVE('',#43036,#43037,#23306,.T.);
#55284=EDGE_CURVE('',#43037,#43038,#1971,.T.);
#55285=EDGE_CURVE('',#43038,#43039,#23307,.T.);
#55286=EDGE_CURVE('',#43039,#43040,#23308,.T.);
#55287=EDGE_CURVE('',#43040,#43041,#1972,.T.);
#55288=EDGE_CURVE('',#43041,#43042,#23309,.T.);
#55289=EDGE_CURVE('',#43042,#43043,#1973,.T.);
#55290=EDGE_CURVE('',#43043,#43044,#23310,.T.);
#55291=EDGE_CURVE('',#43044,#43033,#23311,.T.);
#55292=EDGE_CURVE('',#43045,#43046,#23312,.T.);
#55293=EDGE_CURVE('',#43046,#43047,#34371,.T.);
#55294=EDGE_CURVE('',#43047,#43048,#23313,.T.);
#55295=EDGE_CURVE('',#43048,#43045,#34372,.T.);
#55296=EDGE_CURVE('',#43049,#43050,#1974,.T.);
#55297=EDGE_CURVE('',#43050,#43051,#23314,.T.);
#55298=EDGE_CURVE('',#43051,#43052,#23315,.T.);
#55299=EDGE_CURVE('',#43052,#43053,#23316,.T.);
#55300=EDGE_CURVE('',#43053,#43054,#1975,.T.);
#55301=EDGE_CURVE('',#43054,#43055,#23317,.T.);
#55302=EDGE_CURVE('',#43055,#43056,#23318,.T.);
#55303=EDGE_CURVE('',#43056,#43057,#1976,.T.);
#55304=EDGE_CURVE('',#43057,#43058,#23319,.T.);
#55305=EDGE_CURVE('',#43058,#43059,#1977,.T.);
#55306=EDGE_CURVE('',#43059,#43060,#23320,.T.);
#55307=EDGE_CURVE('',#43060,#43049,#23321,.T.);
#55308=EDGE_CURVE('',#43061,#43062,#1978,.T.);
#55309=EDGE_CURVE('',#43062,#43063,#23322,.T.);
#55310=EDGE_CURVE('',#43063,#43064,#23323,.T.);
#55311=EDGE_CURVE('',#43064,#43065,#23324,.T.);
#55312=EDGE_CURVE('',#43065,#43066,#1979,.T.);
#55313=EDGE_CURVE('',#43066,#43067,#23325,.T.);
#55314=EDGE_CURVE('',#43067,#43068,#23326,.T.);
#55315=EDGE_CURVE('',#43068,#43069,#1980,.T.);
#55316=EDGE_CURVE('',#43069,#43070,#23327,.T.);
#55317=EDGE_CURVE('',#43070,#43071,#1981,.T.);
#55318=EDGE_CURVE('',#43071,#43072,#23328,.T.);
#55319=EDGE_CURVE('',#43072,#43061,#23329,.T.);
#55320=EDGE_CURVE('',#43073,#43074,#23330,.T.);
#55321=EDGE_CURVE('',#43074,#43075,#34373,.T.);
#55322=EDGE_CURVE('',#43075,#43076,#23331,.T.);
#55323=EDGE_CURVE('',#43076,#43073,#34374,.T.);
#55324=EDGE_CURVE('',#43077,#43078,#1982,.T.);
#55325=EDGE_CURVE('',#43078,#43079,#23332,.T.);
#55326=EDGE_CURVE('',#43079,#43080,#23333,.T.);
#55327=EDGE_CURVE('',#43080,#43081,#23334,.T.);
#55328=EDGE_CURVE('',#43081,#43082,#1983,.T.);
#55329=EDGE_CURVE('',#43082,#43083,#23335,.T.);
#55330=EDGE_CURVE('',#43083,#43084,#23336,.T.);
#55331=EDGE_CURVE('',#43084,#43085,#1984,.T.);
#55332=EDGE_CURVE('',#43085,#43086,#23337,.T.);
#55333=EDGE_CURVE('',#43086,#43087,#1985,.T.);
#55334=EDGE_CURVE('',#43087,#43088,#23338,.T.);
#55335=EDGE_CURVE('',#43088,#43077,#23339,.T.);
#55336=EDGE_CURVE('',#43089,#43090,#1986,.T.);
#55337=EDGE_CURVE('',#43090,#43091,#23340,.T.);
#55338=EDGE_CURVE('',#43091,#43092,#23341,.T.);
#55339=EDGE_CURVE('',#43092,#43093,#23342,.T.);
#55340=EDGE_CURVE('',#43093,#43094,#1987,.T.);
#55341=EDGE_CURVE('',#43094,#43095,#23343,.T.);
#55342=EDGE_CURVE('',#43095,#43096,#23344,.T.);
#55343=EDGE_CURVE('',#43096,#43097,#1988,.T.);
#55344=EDGE_CURVE('',#43097,#43098,#23345,.T.);
#55345=EDGE_CURVE('',#43098,#43099,#1989,.T.);
#55346=EDGE_CURVE('',#43099,#43100,#23346,.T.);
#55347=EDGE_CURVE('',#43100,#43089,#23347,.T.);
#55348=EDGE_CURVE('',#43101,#43102,#23348,.T.);
#55349=EDGE_CURVE('',#43102,#43103,#34375,.T.);
#55350=EDGE_CURVE('',#43103,#43104,#23349,.T.);
#55351=EDGE_CURVE('',#43104,#43101,#34376,.T.);
#55352=EDGE_CURVE('',#43105,#43106,#1990,.T.);
#55353=EDGE_CURVE('',#43106,#43107,#23350,.T.);
#55354=EDGE_CURVE('',#43107,#43108,#23351,.T.);
#55355=EDGE_CURVE('',#43108,#43109,#23352,.T.);
#55356=EDGE_CURVE('',#43109,#43110,#1991,.T.);
#55357=EDGE_CURVE('',#43110,#43111,#23353,.T.);
#55358=EDGE_CURVE('',#43111,#43112,#23354,.T.);
#55359=EDGE_CURVE('',#43112,#43113,#1992,.T.);
#55360=EDGE_CURVE('',#43113,#43114,#23355,.T.);
#55361=EDGE_CURVE('',#43114,#43115,#1993,.T.);
#55362=EDGE_CURVE('',#43115,#43116,#23356,.T.);
#55363=EDGE_CURVE('',#43116,#43105,#23357,.T.);
#55364=EDGE_CURVE('',#43117,#43118,#1994,.T.);
#55365=EDGE_CURVE('',#43118,#43119,#23358,.T.);
#55366=EDGE_CURVE('',#43119,#43120,#23359,.T.);
#55367=EDGE_CURVE('',#43120,#43121,#23360,.T.);
#55368=EDGE_CURVE('',#43121,#43122,#1995,.T.);
#55369=EDGE_CURVE('',#43122,#43123,#23361,.T.);
#55370=EDGE_CURVE('',#43123,#43124,#23362,.T.);
#55371=EDGE_CURVE('',#43124,#43125,#1996,.T.);
#55372=EDGE_CURVE('',#43125,#43126,#23363,.T.);
#55373=EDGE_CURVE('',#43126,#43127,#1997,.T.);
#55374=EDGE_CURVE('',#43127,#43128,#23364,.T.);
#55375=EDGE_CURVE('',#43128,#43117,#23365,.T.);
#55376=EDGE_CURVE('',#43129,#43130,#23366,.T.);
#55377=EDGE_CURVE('',#43130,#43131,#34377,.T.);
#55378=EDGE_CURVE('',#43131,#43132,#23367,.T.);
#55379=EDGE_CURVE('',#43132,#43129,#34378,.T.);
#55380=EDGE_CURVE('',#43133,#43134,#1998,.T.);
#55381=EDGE_CURVE('',#43134,#43135,#23368,.T.);
#55382=EDGE_CURVE('',#43135,#43136,#23369,.T.);
#55383=EDGE_CURVE('',#43136,#43137,#23370,.T.);
#55384=EDGE_CURVE('',#43137,#43138,#1999,.T.);
#55385=EDGE_CURVE('',#43138,#43139,#23371,.T.);
#55386=EDGE_CURVE('',#43139,#43140,#23372,.T.);
#55387=EDGE_CURVE('',#43140,#43141,#2000,.T.);
#55388=EDGE_CURVE('',#43141,#43142,#23373,.T.);
#55389=EDGE_CURVE('',#43142,#43143,#2001,.T.);
#55390=EDGE_CURVE('',#43143,#43144,#23374,.T.);
#55391=EDGE_CURVE('',#43144,#43133,#23375,.T.);
#55392=EDGE_CURVE('',#43145,#43146,#2002,.T.);
#55393=EDGE_CURVE('',#43146,#43147,#23376,.T.);
#55394=EDGE_CURVE('',#43147,#43148,#23377,.T.);
#55395=EDGE_CURVE('',#43148,#43149,#23378,.T.);
#55396=EDGE_CURVE('',#43149,#43150,#2003,.T.);
#55397=EDGE_CURVE('',#43150,#43151,#23379,.T.);
#55398=EDGE_CURVE('',#43151,#43152,#23380,.T.);
#55399=EDGE_CURVE('',#43152,#43153,#2004,.T.);
#55400=EDGE_CURVE('',#43153,#43154,#23381,.T.);
#55401=EDGE_CURVE('',#43154,#43155,#2005,.T.);
#55402=EDGE_CURVE('',#43155,#43156,#23382,.T.);
#55403=EDGE_CURVE('',#43156,#43145,#23383,.T.);
#55404=EDGE_CURVE('',#43157,#43158,#23384,.T.);
#55405=EDGE_CURVE('',#43158,#43159,#34379,.T.);
#55406=EDGE_CURVE('',#43159,#43160,#23385,.T.);
#55407=EDGE_CURVE('',#43160,#43157,#34380,.T.);
#55408=EDGE_CURVE('',#43161,#43162,#2006,.T.);
#55409=EDGE_CURVE('',#43162,#43163,#23386,.T.);
#55410=EDGE_CURVE('',#43163,#43164,#23387,.T.);
#55411=EDGE_CURVE('',#43164,#43165,#23388,.T.);
#55412=EDGE_CURVE('',#43165,#43166,#2007,.T.);
#55413=EDGE_CURVE('',#43166,#43167,#23389,.T.);
#55414=EDGE_CURVE('',#43167,#43168,#23390,.T.);
#55415=EDGE_CURVE('',#43168,#43169,#2008,.T.);
#55416=EDGE_CURVE('',#43169,#43170,#23391,.T.);
#55417=EDGE_CURVE('',#43170,#43171,#2009,.T.);
#55418=EDGE_CURVE('',#43171,#43172,#23392,.T.);
#55419=EDGE_CURVE('',#43172,#43161,#23393,.T.);
#55420=EDGE_CURVE('',#43173,#43174,#2010,.T.);
#55421=EDGE_CURVE('',#43174,#43175,#23394,.T.);
#55422=EDGE_CURVE('',#43175,#43176,#23395,.T.);
#55423=EDGE_CURVE('',#43176,#43177,#23396,.T.);
#55424=EDGE_CURVE('',#43177,#43178,#2011,.T.);
#55425=EDGE_CURVE('',#43178,#43179,#23397,.T.);
#55426=EDGE_CURVE('',#43179,#43180,#23398,.T.);
#55427=EDGE_CURVE('',#43180,#43181,#2012,.T.);
#55428=EDGE_CURVE('',#43181,#43182,#23399,.T.);
#55429=EDGE_CURVE('',#43182,#43183,#2013,.T.);
#55430=EDGE_CURVE('',#43183,#43184,#23400,.T.);
#55431=EDGE_CURVE('',#43184,#43173,#23401,.T.);
#55432=EDGE_CURVE('',#43185,#43186,#23402,.T.);
#55433=EDGE_CURVE('',#43186,#43187,#34381,.T.);
#55434=EDGE_CURVE('',#43187,#43188,#23403,.T.);
#55435=EDGE_CURVE('',#43188,#43185,#34382,.T.);
#55436=EDGE_CURVE('',#43189,#43190,#2014,.T.);
#55437=EDGE_CURVE('',#43190,#43191,#23404,.T.);
#55438=EDGE_CURVE('',#43191,#43192,#23405,.T.);
#55439=EDGE_CURVE('',#43192,#43193,#23406,.T.);
#55440=EDGE_CURVE('',#43193,#43194,#2015,.T.);
#55441=EDGE_CURVE('',#43194,#43195,#23407,.T.);
#55442=EDGE_CURVE('',#43195,#43196,#23408,.T.);
#55443=EDGE_CURVE('',#43196,#43197,#2016,.T.);
#55444=EDGE_CURVE('',#43197,#43198,#23409,.T.);
#55445=EDGE_CURVE('',#43198,#43199,#2017,.T.);
#55446=EDGE_CURVE('',#43199,#43200,#23410,.T.);
#55447=EDGE_CURVE('',#43200,#43189,#23411,.T.);
#55448=EDGE_CURVE('',#43201,#43202,#2018,.T.);
#55449=EDGE_CURVE('',#43202,#43203,#23412,.T.);
#55450=EDGE_CURVE('',#43203,#43204,#23413,.T.);
#55451=EDGE_CURVE('',#43204,#43205,#23414,.T.);
#55452=EDGE_CURVE('',#43205,#43206,#2019,.T.);
#55453=EDGE_CURVE('',#43206,#43207,#23415,.T.);
#55454=EDGE_CURVE('',#43207,#43208,#23416,.T.);
#55455=EDGE_CURVE('',#43208,#43209,#2020,.T.);
#55456=EDGE_CURVE('',#43209,#43210,#23417,.T.);
#55457=EDGE_CURVE('',#43210,#43211,#2021,.T.);
#55458=EDGE_CURVE('',#43211,#43212,#23418,.T.);
#55459=EDGE_CURVE('',#43212,#43201,#23419,.T.);
#55460=EDGE_CURVE('',#40437,#40443,#23420,.T.);
#55461=EDGE_CURVE('',#40442,#40436,#23421,.T.);
#55462=EDGE_CURVE('',#43213,#43214,#2022,.T.);
#55463=EDGE_CURVE('',#43214,#43215,#23422,.T.);
#55464=EDGE_CURVE('',#43215,#43216,#23423,.T.);
#55465=EDGE_CURVE('',#43216,#43217,#23424,.T.);
#55466=EDGE_CURVE('',#43217,#43218,#2023,.T.);
#55467=EDGE_CURVE('',#43218,#43219,#23425,.T.);
#55468=EDGE_CURVE('',#43219,#43220,#23426,.T.);
#55469=EDGE_CURVE('',#43220,#43221,#2024,.T.);
#55470=EDGE_CURVE('',#43221,#43222,#23427,.T.);
#55471=EDGE_CURVE('',#43222,#43223,#2025,.T.);
#55472=EDGE_CURVE('',#43223,#43224,#23428,.T.);
#55473=EDGE_CURVE('',#43224,#43213,#23429,.T.);
#55474=EDGE_CURVE('',#43225,#43226,#2026,.T.);
#55475=EDGE_CURVE('',#43226,#43227,#23430,.T.);
#55476=EDGE_CURVE('',#43227,#43228,#23431,.T.);
#55477=EDGE_CURVE('',#43228,#43229,#23432,.T.);
#55478=EDGE_CURVE('',#43229,#43230,#2027,.T.);
#55479=EDGE_CURVE('',#43230,#43231,#23433,.T.);
#55480=EDGE_CURVE('',#43231,#43232,#23434,.T.);
#55481=EDGE_CURVE('',#43232,#43233,#2028,.T.);
#55482=EDGE_CURVE('',#43233,#43234,#23435,.T.);
#55483=EDGE_CURVE('',#43234,#43235,#2029,.T.);
#55484=EDGE_CURVE('',#43235,#43236,#23436,.T.);
#55485=EDGE_CURVE('',#43236,#43225,#23437,.T.);
#55486=EDGE_CURVE('',#43237,#43238,#23438,.T.);
#55487=EDGE_CURVE('',#43238,#43239,#34383,.T.);
#55488=EDGE_CURVE('',#43239,#43240,#23439,.T.);
#55489=EDGE_CURVE('',#43240,#43237,#34384,.T.);
#55490=EDGE_CURVE('',#43241,#43242,#2030,.T.);
#55491=EDGE_CURVE('',#43242,#43243,#23440,.T.);
#55492=EDGE_CURVE('',#43243,#43244,#23441,.T.);
#55493=EDGE_CURVE('',#43244,#43245,#23442,.T.);
#55494=EDGE_CURVE('',#43245,#43246,#2031,.T.);
#55495=EDGE_CURVE('',#43246,#43247,#23443,.T.);
#55496=EDGE_CURVE('',#43247,#43248,#23444,.T.);
#55497=EDGE_CURVE('',#43248,#43249,#2032,.T.);
#55498=EDGE_CURVE('',#43249,#43250,#23445,.T.);
#55499=EDGE_CURVE('',#43250,#43251,#2033,.T.);
#55500=EDGE_CURVE('',#43251,#43252,#23446,.T.);
#55501=EDGE_CURVE('',#43252,#43241,#23447,.T.);
#55502=EDGE_CURVE('',#43253,#43254,#2034,.T.);
#55503=EDGE_CURVE('',#43254,#43255,#23448,.T.);
#55504=EDGE_CURVE('',#43255,#43256,#23449,.T.);
#55505=EDGE_CURVE('',#43256,#43257,#23450,.T.);
#55506=EDGE_CURVE('',#43257,#43258,#2035,.T.);
#55507=EDGE_CURVE('',#43258,#43259,#23451,.T.);
#55508=EDGE_CURVE('',#43259,#43260,#23452,.T.);
#55509=EDGE_CURVE('',#43260,#43261,#2036,.T.);
#55510=EDGE_CURVE('',#43261,#43262,#23453,.T.);
#55511=EDGE_CURVE('',#43262,#43263,#2037,.T.);
#55512=EDGE_CURVE('',#43263,#43264,#23454,.T.);
#55513=EDGE_CURVE('',#43264,#43253,#23455,.T.);
#55514=EDGE_CURVE('',#43265,#43266,#23456,.T.);
#55515=EDGE_CURVE('',#43266,#43267,#34385,.T.);
#55516=EDGE_CURVE('',#43267,#43268,#23457,.T.);
#55517=EDGE_CURVE('',#43268,#43265,#34386,.T.);
#55518=EDGE_CURVE('',#43269,#43270,#2038,.T.);
#55519=EDGE_CURVE('',#43270,#43271,#23458,.T.);
#55520=EDGE_CURVE('',#43271,#43272,#23459,.T.);
#55521=EDGE_CURVE('',#43272,#43273,#23460,.T.);
#55522=EDGE_CURVE('',#43273,#43274,#2039,.T.);
#55523=EDGE_CURVE('',#43274,#43275,#23461,.T.);
#55524=EDGE_CURVE('',#43275,#43276,#23462,.T.);
#55525=EDGE_CURVE('',#43276,#43277,#2040,.T.);
#55526=EDGE_CURVE('',#43277,#43278,#23463,.T.);
#55527=EDGE_CURVE('',#43278,#43279,#2041,.T.);
#55528=EDGE_CURVE('',#43279,#43280,#23464,.T.);
#55529=EDGE_CURVE('',#43280,#43269,#23465,.T.);
#55530=EDGE_CURVE('',#43281,#43282,#2042,.T.);
#55531=EDGE_CURVE('',#43282,#43283,#23466,.T.);
#55532=EDGE_CURVE('',#43283,#43284,#23467,.T.);
#55533=EDGE_CURVE('',#43284,#43285,#23468,.T.);
#55534=EDGE_CURVE('',#43285,#43286,#2043,.T.);
#55535=EDGE_CURVE('',#43286,#43287,#23469,.T.);
#55536=EDGE_CURVE('',#43287,#43288,#23470,.T.);
#55537=EDGE_CURVE('',#43288,#43289,#2044,.T.);
#55538=EDGE_CURVE('',#43289,#43290,#23471,.T.);
#55539=EDGE_CURVE('',#43290,#43291,#2045,.T.);
#55540=EDGE_CURVE('',#43291,#43292,#23472,.T.);
#55541=EDGE_CURVE('',#43292,#43281,#23473,.T.);
#55542=EDGE_CURVE('',#43293,#43294,#23474,.T.);
#55543=EDGE_CURVE('',#43294,#43295,#34387,.T.);
#55544=EDGE_CURVE('',#43295,#43296,#23475,.T.);
#55545=EDGE_CURVE('',#43296,#43293,#34388,.T.);
#55546=EDGE_CURVE('',#43297,#43298,#2046,.T.);
#55547=EDGE_CURVE('',#43298,#43299,#23476,.T.);
#55548=EDGE_CURVE('',#43299,#43300,#23477,.T.);
#55549=EDGE_CURVE('',#43300,#43301,#23478,.T.);
#55550=EDGE_CURVE('',#43301,#43302,#2047,.T.);
#55551=EDGE_CURVE('',#43302,#43303,#23479,.T.);
#55552=EDGE_CURVE('',#43303,#43304,#23480,.T.);
#55553=EDGE_CURVE('',#43304,#43305,#2048,.T.);
#55554=EDGE_CURVE('',#43305,#43306,#23481,.T.);
#55555=EDGE_CURVE('',#43306,#43307,#2049,.T.);
#55556=EDGE_CURVE('',#43307,#43308,#23482,.T.);
#55557=EDGE_CURVE('',#43308,#43297,#23483,.T.);
#55558=EDGE_CURVE('',#43309,#43310,#2050,.T.);
#55559=EDGE_CURVE('',#43310,#43311,#23484,.T.);
#55560=EDGE_CURVE('',#43311,#43312,#23485,.T.);
#55561=EDGE_CURVE('',#43312,#43313,#23486,.T.);
#55562=EDGE_CURVE('',#43313,#43314,#2051,.T.);
#55563=EDGE_CURVE('',#43314,#43315,#23487,.T.);
#55564=EDGE_CURVE('',#43315,#43316,#23488,.T.);
#55565=EDGE_CURVE('',#43316,#43317,#2052,.T.);
#55566=EDGE_CURVE('',#43317,#43318,#23489,.T.);
#55567=EDGE_CURVE('',#43318,#43319,#2053,.T.);
#55568=EDGE_CURVE('',#43319,#43320,#23490,.T.);
#55569=EDGE_CURVE('',#43320,#43309,#23491,.T.);
#55570=EDGE_CURVE('',#43321,#43322,#23492,.T.);
#55571=EDGE_CURVE('',#43322,#43323,#34389,.T.);
#55572=EDGE_CURVE('',#43323,#43324,#23493,.T.);
#55573=EDGE_CURVE('',#43324,#43321,#34390,.T.);
#55574=EDGE_CURVE('',#43325,#43326,#2054,.T.);
#55575=EDGE_CURVE('',#43326,#43327,#23494,.T.);
#55576=EDGE_CURVE('',#43327,#43328,#23495,.T.);
#55577=EDGE_CURVE('',#43328,#43329,#23496,.T.);
#55578=EDGE_CURVE('',#43329,#43330,#2055,.T.);
#55579=EDGE_CURVE('',#43330,#43331,#23497,.T.);
#55580=EDGE_CURVE('',#43331,#43332,#23498,.T.);
#55581=EDGE_CURVE('',#43332,#43333,#2056,.T.);
#55582=EDGE_CURVE('',#43333,#43334,#23499,.T.);
#55583=EDGE_CURVE('',#43334,#43335,#2057,.T.);
#55584=EDGE_CURVE('',#43335,#43336,#23500,.T.);
#55585=EDGE_CURVE('',#43336,#43325,#23501,.T.);
#55586=EDGE_CURVE('',#43337,#43338,#2058,.T.);
#55587=EDGE_CURVE('',#43338,#43339,#23502,.T.);
#55588=EDGE_CURVE('',#43339,#43340,#23503,.T.);
#55589=EDGE_CURVE('',#43340,#43341,#23504,.T.);
#55590=EDGE_CURVE('',#43341,#43342,#2059,.T.);
#55591=EDGE_CURVE('',#43342,#43343,#23505,.T.);
#55592=EDGE_CURVE('',#43343,#43344,#23506,.T.);
#55593=EDGE_CURVE('',#43344,#43345,#2060,.T.);
#55594=EDGE_CURVE('',#43345,#43346,#23507,.T.);
#55595=EDGE_CURVE('',#43346,#43347,#2061,.T.);
#55596=EDGE_CURVE('',#43347,#43348,#23508,.T.);
#55597=EDGE_CURVE('',#43348,#43337,#23509,.T.);
#55598=EDGE_CURVE('',#43349,#43350,#23510,.T.);
#55599=EDGE_CURVE('',#43350,#43351,#34391,.T.);
#55600=EDGE_CURVE('',#43351,#43352,#23511,.T.);
#55601=EDGE_CURVE('',#43352,#43349,#34392,.T.);
#55602=EDGE_CURVE('',#43353,#43354,#2062,.T.);
#55603=EDGE_CURVE('',#43354,#43355,#23512,.T.);
#55604=EDGE_CURVE('',#43355,#43356,#23513,.T.);
#55605=EDGE_CURVE('',#43356,#43357,#23514,.T.);
#55606=EDGE_CURVE('',#43357,#43358,#2063,.T.);
#55607=EDGE_CURVE('',#43358,#43359,#23515,.T.);
#55608=EDGE_CURVE('',#43359,#43360,#23516,.T.);
#55609=EDGE_CURVE('',#43360,#43361,#2064,.T.);
#55610=EDGE_CURVE('',#43361,#43362,#23517,.T.);
#55611=EDGE_CURVE('',#43362,#43363,#2065,.T.);
#55612=EDGE_CURVE('',#43363,#43364,#23518,.T.);
#55613=EDGE_CURVE('',#43364,#43353,#23519,.T.);
#55614=EDGE_CURVE('',#43365,#43366,#2066,.T.);
#55615=EDGE_CURVE('',#43366,#43367,#23520,.T.);
#55616=EDGE_CURVE('',#43367,#43368,#23521,.T.);
#55617=EDGE_CURVE('',#43368,#43369,#23522,.T.);
#55618=EDGE_CURVE('',#43369,#43370,#2067,.T.);
#55619=EDGE_CURVE('',#43370,#43371,#23523,.T.);
#55620=EDGE_CURVE('',#43371,#43372,#23524,.T.);
#55621=EDGE_CURVE('',#43372,#43373,#2068,.T.);
#55622=EDGE_CURVE('',#43373,#43374,#23525,.T.);
#55623=EDGE_CURVE('',#43374,#43375,#2069,.T.);
#55624=EDGE_CURVE('',#43375,#43376,#23526,.T.);
#55625=EDGE_CURVE('',#43376,#43365,#23527,.T.);
#55626=EDGE_CURVE('',#43377,#43378,#23528,.T.);
#55627=EDGE_CURVE('',#43378,#43379,#34393,.T.);
#55628=EDGE_CURVE('',#43379,#43380,#23529,.T.);
#55629=EDGE_CURVE('',#43380,#43377,#34394,.T.);
#55630=EDGE_CURVE('',#43381,#43382,#2070,.T.);
#55631=EDGE_CURVE('',#43382,#43383,#23530,.T.);
#55632=EDGE_CURVE('',#43383,#43384,#23531,.T.);
#55633=EDGE_CURVE('',#43384,#43385,#23532,.T.);
#55634=EDGE_CURVE('',#43385,#43386,#2071,.T.);
#55635=EDGE_CURVE('',#43386,#43387,#23533,.T.);
#55636=EDGE_CURVE('',#43387,#43388,#23534,.T.);
#55637=EDGE_CURVE('',#43388,#43389,#2072,.T.);
#55638=EDGE_CURVE('',#43389,#43390,#23535,.T.);
#55639=EDGE_CURVE('',#43390,#43391,#2073,.T.);
#55640=EDGE_CURVE('',#43391,#43392,#23536,.T.);
#55641=EDGE_CURVE('',#43392,#43381,#23537,.T.);
#55642=EDGE_CURVE('',#43393,#43394,#2074,.T.);
#55643=EDGE_CURVE('',#43394,#43395,#23538,.T.);
#55644=EDGE_CURVE('',#43395,#43396,#23539,.T.);
#55645=EDGE_CURVE('',#43396,#43397,#23540,.T.);
#55646=EDGE_CURVE('',#43397,#43398,#2075,.T.);
#55647=EDGE_CURVE('',#43398,#43399,#23541,.T.);
#55648=EDGE_CURVE('',#43399,#43400,#23542,.T.);
#55649=EDGE_CURVE('',#43400,#43401,#2076,.T.);
#55650=EDGE_CURVE('',#43401,#43402,#23543,.T.);
#55651=EDGE_CURVE('',#43402,#43403,#2077,.T.);
#55652=EDGE_CURVE('',#43403,#43404,#23544,.T.);
#55653=EDGE_CURVE('',#43404,#43393,#23545,.T.);
#55654=EDGE_CURVE('',#43405,#43406,#23546,.T.);
#55655=EDGE_CURVE('',#43406,#43407,#34395,.T.);
#55656=EDGE_CURVE('',#43407,#43408,#23547,.T.);
#55657=EDGE_CURVE('',#43408,#43405,#34396,.T.);
#55658=EDGE_CURVE('',#43409,#43410,#2078,.T.);
#55659=EDGE_CURVE('',#43410,#43411,#23548,.T.);
#55660=EDGE_CURVE('',#43411,#43412,#23549,.T.);
#55661=EDGE_CURVE('',#43412,#43413,#23550,.T.);
#55662=EDGE_CURVE('',#43413,#43414,#2079,.T.);
#55663=EDGE_CURVE('',#43414,#43415,#23551,.T.);
#55664=EDGE_CURVE('',#43415,#43416,#23552,.T.);
#55665=EDGE_CURVE('',#43416,#43417,#2080,.T.);
#55666=EDGE_CURVE('',#43417,#43418,#23553,.T.);
#55667=EDGE_CURVE('',#43418,#43419,#2081,.T.);
#55668=EDGE_CURVE('',#43419,#43420,#23554,.T.);
#55669=EDGE_CURVE('',#43420,#43409,#23555,.T.);
#55670=EDGE_CURVE('',#43421,#43422,#2082,.T.);
#55671=EDGE_CURVE('',#43422,#43423,#23556,.T.);
#55672=EDGE_CURVE('',#43423,#43424,#23557,.T.);
#55673=EDGE_CURVE('',#43424,#43425,#23558,.T.);
#55674=EDGE_CURVE('',#43425,#43426,#2083,.T.);
#55675=EDGE_CURVE('',#43426,#43427,#23559,.T.);
#55676=EDGE_CURVE('',#43427,#43428,#23560,.T.);
#55677=EDGE_CURVE('',#43428,#43429,#2084,.T.);
#55678=EDGE_CURVE('',#43429,#43430,#23561,.T.);
#55679=EDGE_CURVE('',#43430,#43431,#2085,.T.);
#55680=EDGE_CURVE('',#43431,#43432,#23562,.T.);
#55681=EDGE_CURVE('',#43432,#43421,#23563,.T.);
#55682=EDGE_CURVE('',#43433,#43434,#23564,.T.);
#55683=EDGE_CURVE('',#43434,#43435,#34397,.T.);
#55684=EDGE_CURVE('',#43435,#43436,#23565,.T.);
#55685=EDGE_CURVE('',#43436,#43433,#34398,.T.);
#55686=EDGE_CURVE('',#43437,#43438,#2086,.T.);
#55687=EDGE_CURVE('',#43438,#43439,#23566,.T.);
#55688=EDGE_CURVE('',#43439,#43440,#23567,.T.);
#55689=EDGE_CURVE('',#43440,#43441,#23568,.T.);
#55690=EDGE_CURVE('',#43441,#43442,#2087,.T.);
#55691=EDGE_CURVE('',#43442,#43443,#23569,.T.);
#55692=EDGE_CURVE('',#43443,#43444,#23570,.T.);
#55693=EDGE_CURVE('',#43444,#43445,#2088,.T.);
#55694=EDGE_CURVE('',#43445,#43446,#23571,.T.);
#55695=EDGE_CURVE('',#43446,#43447,#2089,.T.);
#55696=EDGE_CURVE('',#43447,#43448,#23572,.T.);
#55697=EDGE_CURVE('',#43448,#43437,#23573,.T.);
#55698=EDGE_CURVE('',#43449,#43450,#2090,.T.);
#55699=EDGE_CURVE('',#43450,#43451,#23574,.T.);
#55700=EDGE_CURVE('',#43451,#43452,#23575,.T.);
#55701=EDGE_CURVE('',#43452,#43453,#23576,.T.);
#55702=EDGE_CURVE('',#43453,#43454,#2091,.T.);
#55703=EDGE_CURVE('',#43454,#43455,#23577,.T.);
#55704=EDGE_CURVE('',#43455,#43456,#23578,.T.);
#55705=EDGE_CURVE('',#43456,#43457,#2092,.T.);
#55706=EDGE_CURVE('',#43457,#43458,#23579,.T.);
#55707=EDGE_CURVE('',#43458,#43459,#2093,.T.);
#55708=EDGE_CURVE('',#43459,#43460,#23580,.T.);
#55709=EDGE_CURVE('',#43460,#43449,#23581,.T.);
#55710=EDGE_CURVE('',#43461,#43462,#23582,.T.);
#55711=EDGE_CURVE('',#43462,#43463,#34399,.T.);
#55712=EDGE_CURVE('',#43463,#43464,#23583,.T.);
#55713=EDGE_CURVE('',#43464,#43461,#34400,.T.);
#55714=EDGE_CURVE('',#43465,#43466,#2094,.T.);
#55715=EDGE_CURVE('',#43466,#43467,#23584,.T.);
#55716=EDGE_CURVE('',#43467,#43468,#23585,.T.);
#55717=EDGE_CURVE('',#43468,#43469,#23586,.T.);
#55718=EDGE_CURVE('',#43469,#43470,#2095,.T.);
#55719=EDGE_CURVE('',#43470,#43471,#23587,.T.);
#55720=EDGE_CURVE('',#43471,#43472,#23588,.T.);
#55721=EDGE_CURVE('',#43472,#43473,#2096,.T.);
#55722=EDGE_CURVE('',#43473,#43474,#23589,.T.);
#55723=EDGE_CURVE('',#43474,#43475,#2097,.T.);
#55724=EDGE_CURVE('',#43475,#43476,#23590,.T.);
#55725=EDGE_CURVE('',#43476,#43465,#23591,.T.);
#55726=EDGE_CURVE('',#43477,#43478,#2098,.T.);
#55727=EDGE_CURVE('',#43478,#43479,#23592,.T.);
#55728=EDGE_CURVE('',#43479,#43480,#23593,.T.);
#55729=EDGE_CURVE('',#43480,#43481,#23594,.T.);
#55730=EDGE_CURVE('',#43481,#43482,#2099,.T.);
#55731=EDGE_CURVE('',#43482,#43483,#23595,.T.);
#55732=EDGE_CURVE('',#43483,#43484,#23596,.T.);
#55733=EDGE_CURVE('',#43484,#43485,#2100,.T.);
#55734=EDGE_CURVE('',#43485,#43486,#23597,.T.);
#55735=EDGE_CURVE('',#43486,#43487,#2101,.T.);
#55736=EDGE_CURVE('',#43487,#43488,#23598,.T.);
#55737=EDGE_CURVE('',#43488,#43477,#23599,.T.);
#55738=EDGE_CURVE('',#43489,#43490,#23600,.T.);
#55739=EDGE_CURVE('',#43490,#43491,#34401,.T.);
#55740=EDGE_CURVE('',#43491,#43492,#23601,.T.);
#55741=EDGE_CURVE('',#43492,#43489,#34402,.T.);
#55742=EDGE_CURVE('',#43493,#43494,#2102,.T.);
#55743=EDGE_CURVE('',#43494,#43495,#23602,.T.);
#55744=EDGE_CURVE('',#43495,#43496,#23603,.T.);
#55745=EDGE_CURVE('',#43496,#43497,#23604,.T.);
#55746=EDGE_CURVE('',#43497,#43498,#2103,.T.);
#55747=EDGE_CURVE('',#43498,#43499,#23605,.T.);
#55748=EDGE_CURVE('',#43499,#43500,#23606,.T.);
#55749=EDGE_CURVE('',#43500,#43501,#2104,.T.);
#55750=EDGE_CURVE('',#43501,#43502,#23607,.T.);
#55751=EDGE_CURVE('',#43502,#43503,#2105,.T.);
#55752=EDGE_CURVE('',#43503,#43504,#23608,.T.);
#55753=EDGE_CURVE('',#43504,#43493,#23609,.T.);
#55754=EDGE_CURVE('',#43505,#43506,#2106,.T.);
#55755=EDGE_CURVE('',#43506,#43507,#23610,.T.);
#55756=EDGE_CURVE('',#43507,#43508,#23611,.T.);
#55757=EDGE_CURVE('',#43508,#43509,#23612,.T.);
#55758=EDGE_CURVE('',#43509,#43510,#2107,.T.);
#55759=EDGE_CURVE('',#43510,#43511,#23613,.T.);
#55760=EDGE_CURVE('',#43511,#43512,#23614,.T.);
#55761=EDGE_CURVE('',#43512,#43513,#2108,.T.);
#55762=EDGE_CURVE('',#43513,#43514,#23615,.T.);
#55763=EDGE_CURVE('',#43514,#43515,#2109,.T.);
#55764=EDGE_CURVE('',#43515,#43516,#23616,.T.);
#55765=EDGE_CURVE('',#43516,#43505,#23617,.T.);
#55766=EDGE_CURVE('',#43517,#43518,#23618,.T.);
#55767=EDGE_CURVE('',#43518,#43519,#34403,.T.);
#55768=EDGE_CURVE('',#43519,#43520,#23619,.T.);
#55769=EDGE_CURVE('',#43520,#43517,#34404,.T.);
#55770=EDGE_CURVE('',#43521,#43522,#2110,.T.);
#55771=EDGE_CURVE('',#43522,#43523,#23620,.T.);
#55772=EDGE_CURVE('',#43523,#43524,#23621,.T.);
#55773=EDGE_CURVE('',#43524,#43525,#23622,.T.);
#55774=EDGE_CURVE('',#43525,#43526,#2111,.T.);
#55775=EDGE_CURVE('',#43526,#43527,#23623,.T.);
#55776=EDGE_CURVE('',#43527,#43528,#23624,.T.);
#55777=EDGE_CURVE('',#43528,#43529,#2112,.T.);
#55778=EDGE_CURVE('',#43529,#43530,#23625,.T.);
#55779=EDGE_CURVE('',#43530,#43531,#2113,.T.);
#55780=EDGE_CURVE('',#43531,#43532,#23626,.T.);
#55781=EDGE_CURVE('',#43532,#43521,#23627,.T.);
#55782=EDGE_CURVE('',#43533,#43534,#2114,.T.);
#55783=EDGE_CURVE('',#43534,#43535,#23628,.T.);
#55784=EDGE_CURVE('',#43535,#43536,#23629,.T.);
#55785=EDGE_CURVE('',#43536,#43537,#23630,.T.);
#55786=EDGE_CURVE('',#43537,#43538,#2115,.T.);
#55787=EDGE_CURVE('',#43538,#43539,#23631,.T.);
#55788=EDGE_CURVE('',#43539,#43540,#23632,.T.);
#55789=EDGE_CURVE('',#43540,#43541,#2116,.T.);
#55790=EDGE_CURVE('',#43541,#43542,#23633,.T.);
#55791=EDGE_CURVE('',#43542,#43543,#2117,.T.);
#55792=EDGE_CURVE('',#43543,#43544,#23634,.T.);
#55793=EDGE_CURVE('',#43544,#43533,#23635,.T.);
#55794=EDGE_CURVE('',#43545,#43546,#23636,.T.);
#55795=EDGE_CURVE('',#43546,#43547,#34405,.T.);
#55796=EDGE_CURVE('',#43547,#43548,#23637,.T.);
#55797=EDGE_CURVE('',#43548,#43545,#34406,.T.);
#55798=EDGE_CURVE('',#43549,#43550,#2118,.T.);
#55799=EDGE_CURVE('',#43550,#43551,#23638,.T.);
#55800=EDGE_CURVE('',#43551,#43552,#23639,.T.);
#55801=EDGE_CURVE('',#43552,#43553,#23640,.T.);
#55802=EDGE_CURVE('',#43553,#43554,#2119,.T.);
#55803=EDGE_CURVE('',#43554,#43555,#23641,.T.);
#55804=EDGE_CURVE('',#43555,#43556,#23642,.T.);
#55805=EDGE_CURVE('',#43556,#43557,#2120,.T.);
#55806=EDGE_CURVE('',#43557,#43558,#23643,.T.);
#55807=EDGE_CURVE('',#43558,#43559,#2121,.T.);
#55808=EDGE_CURVE('',#43559,#43560,#23644,.T.);
#55809=EDGE_CURVE('',#43560,#43549,#23645,.T.);
#55810=EDGE_CURVE('',#43561,#43562,#2122,.T.);
#55811=EDGE_CURVE('',#43562,#43563,#23646,.T.);
#55812=EDGE_CURVE('',#43563,#43564,#23647,.T.);
#55813=EDGE_CURVE('',#43564,#43565,#23648,.T.);
#55814=EDGE_CURVE('',#43565,#43566,#2123,.T.);
#55815=EDGE_CURVE('',#43566,#43567,#23649,.T.);
#55816=EDGE_CURVE('',#43567,#43568,#23650,.T.);
#55817=EDGE_CURVE('',#43568,#43569,#2124,.T.);
#55818=EDGE_CURVE('',#43569,#43570,#23651,.T.);
#55819=EDGE_CURVE('',#43570,#43571,#2125,.T.);
#55820=EDGE_CURVE('',#43571,#43572,#23652,.T.);
#55821=EDGE_CURVE('',#43572,#43561,#23653,.T.);
#55822=EDGE_CURVE('',#43573,#43574,#23654,.T.);
#55823=EDGE_CURVE('',#43574,#43575,#34407,.T.);
#55824=EDGE_CURVE('',#43575,#43576,#23655,.T.);
#55825=EDGE_CURVE('',#43576,#43573,#34408,.T.);
#55826=EDGE_CURVE('',#43577,#43578,#2126,.T.);
#55827=EDGE_CURVE('',#43578,#43579,#23656,.T.);
#55828=EDGE_CURVE('',#43579,#43580,#23657,.T.);
#55829=EDGE_CURVE('',#43580,#43581,#23658,.T.);
#55830=EDGE_CURVE('',#43581,#43582,#2127,.T.);
#55831=EDGE_CURVE('',#43582,#43583,#23659,.T.);
#55832=EDGE_CURVE('',#43583,#43584,#23660,.T.);
#55833=EDGE_CURVE('',#43584,#43585,#2128,.T.);
#55834=EDGE_CURVE('',#43585,#43586,#23661,.T.);
#55835=EDGE_CURVE('',#43586,#43587,#2129,.T.);
#55836=EDGE_CURVE('',#43587,#43588,#23662,.T.);
#55837=EDGE_CURVE('',#43588,#43577,#23663,.T.);
#55838=EDGE_CURVE('',#43589,#43590,#2130,.T.);
#55839=EDGE_CURVE('',#43590,#43591,#23664,.T.);
#55840=EDGE_CURVE('',#43591,#43592,#23665,.T.);
#55841=EDGE_CURVE('',#43592,#43593,#23666,.T.);
#55842=EDGE_CURVE('',#43593,#43594,#2131,.T.);
#55843=EDGE_CURVE('',#43594,#43595,#23667,.T.);
#55844=EDGE_CURVE('',#43595,#43596,#23668,.T.);
#55845=EDGE_CURVE('',#43596,#43597,#2132,.T.);
#55846=EDGE_CURVE('',#43597,#43598,#23669,.T.);
#55847=EDGE_CURVE('',#43598,#43599,#2133,.T.);
#55848=EDGE_CURVE('',#43599,#43600,#23670,.T.);
#55849=EDGE_CURVE('',#43600,#43589,#23671,.T.);
#55850=EDGE_CURVE('',#43601,#43602,#23672,.T.);
#55851=EDGE_CURVE('',#43602,#43603,#34409,.T.);
#55852=EDGE_CURVE('',#43603,#43604,#23673,.T.);
#55853=EDGE_CURVE('',#43604,#43601,#34410,.T.);
#55854=EDGE_CURVE('',#43605,#43606,#2134,.T.);
#55855=EDGE_CURVE('',#43606,#43607,#23674,.T.);
#55856=EDGE_CURVE('',#43607,#43608,#23675,.T.);
#55857=EDGE_CURVE('',#43608,#43609,#23676,.T.);
#55858=EDGE_CURVE('',#43609,#43610,#2135,.T.);
#55859=EDGE_CURVE('',#43610,#43611,#23677,.T.);
#55860=EDGE_CURVE('',#43611,#43612,#23678,.T.);
#55861=EDGE_CURVE('',#43612,#43613,#2136,.T.);
#55862=EDGE_CURVE('',#43613,#43614,#23679,.T.);
#55863=EDGE_CURVE('',#43614,#43615,#2137,.T.);
#55864=EDGE_CURVE('',#43615,#43616,#23680,.T.);
#55865=EDGE_CURVE('',#43616,#43605,#23681,.T.);
#55866=EDGE_CURVE('',#43617,#43618,#2138,.T.);
#55867=EDGE_CURVE('',#43618,#43619,#23682,.T.);
#55868=EDGE_CURVE('',#43619,#43620,#23683,.T.);
#55869=EDGE_CURVE('',#43620,#43621,#23684,.T.);
#55870=EDGE_CURVE('',#43621,#43622,#2139,.T.);
#55871=EDGE_CURVE('',#43622,#43623,#23685,.T.);
#55872=EDGE_CURVE('',#43623,#43624,#23686,.T.);
#55873=EDGE_CURVE('',#43624,#43625,#2140,.T.);
#55874=EDGE_CURVE('',#43625,#43626,#23687,.T.);
#55875=EDGE_CURVE('',#43626,#43627,#2141,.T.);
#55876=EDGE_CURVE('',#43627,#43628,#23688,.T.);
#55877=EDGE_CURVE('',#43628,#43617,#23689,.T.);
#55878=EDGE_CURVE('',#40429,#40435,#23690,.T.);
#55879=EDGE_CURVE('',#40434,#40428,#23691,.T.);
#55880=EDGE_CURVE('',#43629,#43630,#2142,.T.);
#55881=EDGE_CURVE('',#43630,#43631,#23692,.T.);
#55882=EDGE_CURVE('',#43631,#43632,#23693,.T.);
#55883=EDGE_CURVE('',#43632,#43633,#23694,.T.);
#55884=EDGE_CURVE('',#43633,#43634,#2143,.T.);
#55885=EDGE_CURVE('',#43634,#43635,#23695,.T.);
#55886=EDGE_CURVE('',#43635,#43636,#23696,.T.);
#55887=EDGE_CURVE('',#43636,#43637,#2144,.T.);
#55888=EDGE_CURVE('',#43637,#43638,#23697,.T.);
#55889=EDGE_CURVE('',#43638,#43639,#2145,.T.);
#55890=EDGE_CURVE('',#43639,#43640,#23698,.T.);
#55891=EDGE_CURVE('',#43640,#43629,#23699,.T.);
#55892=EDGE_CURVE('',#43641,#43642,#2146,.T.);
#55893=EDGE_CURVE('',#43642,#43643,#23700,.T.);
#55894=EDGE_CURVE('',#43643,#43644,#23701,.T.);
#55895=EDGE_CURVE('',#43644,#43645,#23702,.T.);
#55896=EDGE_CURVE('',#43645,#43646,#2147,.T.);
#55897=EDGE_CURVE('',#43646,#43647,#23703,.T.);
#55898=EDGE_CURVE('',#43647,#43648,#23704,.T.);
#55899=EDGE_CURVE('',#43648,#43649,#2148,.T.);
#55900=EDGE_CURVE('',#43649,#43650,#23705,.T.);
#55901=EDGE_CURVE('',#43650,#43651,#2149,.T.);
#55902=EDGE_CURVE('',#43651,#43652,#23706,.T.);
#55903=EDGE_CURVE('',#43652,#43641,#23707,.T.);
#55904=EDGE_CURVE('',#43653,#43654,#23708,.T.);
#55905=EDGE_CURVE('',#43654,#43655,#34411,.T.);
#55906=EDGE_CURVE('',#43655,#43656,#23709,.T.);
#55907=EDGE_CURVE('',#43656,#43653,#34412,.T.);
#55908=EDGE_CURVE('',#43657,#43658,#2150,.T.);
#55909=EDGE_CURVE('',#43658,#43659,#23710,.T.);
#55910=EDGE_CURVE('',#43659,#43660,#23711,.T.);
#55911=EDGE_CURVE('',#43660,#43661,#23712,.T.);
#55912=EDGE_CURVE('',#43661,#43662,#2151,.T.);
#55913=EDGE_CURVE('',#43662,#43663,#23713,.T.);
#55914=EDGE_CURVE('',#43663,#43664,#23714,.T.);
#55915=EDGE_CURVE('',#43664,#43665,#2152,.T.);
#55916=EDGE_CURVE('',#43665,#43666,#23715,.T.);
#55917=EDGE_CURVE('',#43666,#43667,#2153,.T.);
#55918=EDGE_CURVE('',#43667,#43668,#23716,.T.);
#55919=EDGE_CURVE('',#43668,#43657,#23717,.T.);
#55920=EDGE_CURVE('',#43669,#43670,#2154,.T.);
#55921=EDGE_CURVE('',#43670,#43671,#23718,.T.);
#55922=EDGE_CURVE('',#43671,#43672,#23719,.T.);
#55923=EDGE_CURVE('',#43672,#43673,#23720,.T.);
#55924=EDGE_CURVE('',#43673,#43674,#2155,.T.);
#55925=EDGE_CURVE('',#43674,#43675,#23721,.T.);
#55926=EDGE_CURVE('',#43675,#43676,#23722,.T.);
#55927=EDGE_CURVE('',#43676,#43677,#2156,.T.);
#55928=EDGE_CURVE('',#43677,#43678,#23723,.T.);
#55929=EDGE_CURVE('',#43678,#43679,#2157,.T.);
#55930=EDGE_CURVE('',#43679,#43680,#23724,.T.);
#55931=EDGE_CURVE('',#43680,#43669,#23725,.T.);
#55932=EDGE_CURVE('',#43681,#43682,#23726,.T.);
#55933=EDGE_CURVE('',#43682,#43683,#34413,.T.);
#55934=EDGE_CURVE('',#43683,#43684,#23727,.T.);
#55935=EDGE_CURVE('',#43684,#43681,#34414,.T.);
#55936=EDGE_CURVE('',#43685,#43686,#2158,.T.);
#55937=EDGE_CURVE('',#43686,#43687,#23728,.T.);
#55938=EDGE_CURVE('',#43687,#43688,#23729,.T.);
#55939=EDGE_CURVE('',#43688,#43689,#23730,.T.);
#55940=EDGE_CURVE('',#43689,#43690,#2159,.T.);
#55941=EDGE_CURVE('',#43690,#43691,#23731,.T.);
#55942=EDGE_CURVE('',#43691,#43692,#23732,.T.);
#55943=EDGE_CURVE('',#43692,#43693,#2160,.T.);
#55944=EDGE_CURVE('',#43693,#43694,#23733,.T.);
#55945=EDGE_CURVE('',#43694,#43695,#2161,.T.);
#55946=EDGE_CURVE('',#43695,#43696,#23734,.T.);
#55947=EDGE_CURVE('',#43696,#43685,#23735,.T.);
#55948=EDGE_CURVE('',#43697,#43698,#2162,.T.);
#55949=EDGE_CURVE('',#43698,#43699,#23736,.T.);
#55950=EDGE_CURVE('',#43699,#43700,#23737,.T.);
#55951=EDGE_CURVE('',#43700,#43701,#23738,.T.);
#55952=EDGE_CURVE('',#43701,#43702,#2163,.T.);
#55953=EDGE_CURVE('',#43702,#43703,#23739,.T.);
#55954=EDGE_CURVE('',#43703,#43704,#23740,.T.);
#55955=EDGE_CURVE('',#43704,#43705,#2164,.T.);
#55956=EDGE_CURVE('',#43705,#43706,#23741,.T.);
#55957=EDGE_CURVE('',#43706,#43707,#2165,.T.);
#55958=EDGE_CURVE('',#43707,#43708,#23742,.T.);
#55959=EDGE_CURVE('',#43708,#43697,#23743,.T.);
#55960=EDGE_CURVE('',#43709,#43710,#23744,.T.);
#55961=EDGE_CURVE('',#43710,#43711,#34415,.T.);
#55962=EDGE_CURVE('',#43711,#43712,#23745,.T.);
#55963=EDGE_CURVE('',#43712,#43709,#34416,.T.);
#55964=EDGE_CURVE('',#43713,#43714,#2166,.T.);
#55965=EDGE_CURVE('',#43714,#43715,#23746,.T.);
#55966=EDGE_CURVE('',#43715,#43716,#23747,.T.);
#55967=EDGE_CURVE('',#43716,#43717,#23748,.T.);
#55968=EDGE_CURVE('',#43717,#43718,#2167,.T.);
#55969=EDGE_CURVE('',#43718,#43719,#23749,.T.);
#55970=EDGE_CURVE('',#43719,#43720,#23750,.T.);
#55971=EDGE_CURVE('',#43720,#43721,#2168,.T.);
#55972=EDGE_CURVE('',#43721,#43722,#23751,.T.);
#55973=EDGE_CURVE('',#43722,#43723,#2169,.T.);
#55974=EDGE_CURVE('',#43723,#43724,#23752,.T.);
#55975=EDGE_CURVE('',#43724,#43713,#23753,.T.);
#55976=EDGE_CURVE('',#43725,#43726,#2170,.T.);
#55977=EDGE_CURVE('',#43726,#43727,#23754,.T.);
#55978=EDGE_CURVE('',#43727,#43728,#23755,.T.);
#55979=EDGE_CURVE('',#43728,#43729,#23756,.T.);
#55980=EDGE_CURVE('',#43729,#43730,#2171,.T.);
#55981=EDGE_CURVE('',#43730,#43731,#23757,.T.);
#55982=EDGE_CURVE('',#43731,#43732,#23758,.T.);
#55983=EDGE_CURVE('',#43732,#43733,#2172,.T.);
#55984=EDGE_CURVE('',#43733,#43734,#23759,.T.);
#55985=EDGE_CURVE('',#43734,#43735,#2173,.T.);
#55986=EDGE_CURVE('',#43735,#43736,#23760,.T.);
#55987=EDGE_CURVE('',#43736,#43725,#23761,.T.);
#55988=EDGE_CURVE('',#43737,#43738,#23762,.T.);
#55989=EDGE_CURVE('',#43738,#43739,#34417,.T.);
#55990=EDGE_CURVE('',#43739,#43740,#23763,.T.);
#55991=EDGE_CURVE('',#43740,#43737,#34418,.T.);
#55992=EDGE_CURVE('',#43741,#43742,#2174,.T.);
#55993=EDGE_CURVE('',#43742,#43743,#23764,.T.);
#55994=EDGE_CURVE('',#43743,#43744,#23765,.T.);
#55995=EDGE_CURVE('',#43744,#43745,#23766,.T.);
#55996=EDGE_CURVE('',#43745,#43746,#2175,.T.);
#55997=EDGE_CURVE('',#43746,#43747,#23767,.T.);
#55998=EDGE_CURVE('',#43747,#43748,#23768,.T.);
#55999=EDGE_CURVE('',#43748,#43749,#2176,.T.);
#56000=EDGE_CURVE('',#43749,#43750,#23769,.T.);
#56001=EDGE_CURVE('',#43750,#43751,#2177,.T.);
#56002=EDGE_CURVE('',#43751,#43752,#23770,.T.);
#56003=EDGE_CURVE('',#43752,#43741,#23771,.T.);
#56004=EDGE_CURVE('',#43753,#43754,#2178,.T.);
#56005=EDGE_CURVE('',#43754,#43755,#23772,.T.);
#56006=EDGE_CURVE('',#43755,#43756,#23773,.T.);
#56007=EDGE_CURVE('',#43756,#43757,#23774,.T.);
#56008=EDGE_CURVE('',#43757,#43758,#2179,.T.);
#56009=EDGE_CURVE('',#43758,#43759,#23775,.T.);
#56010=EDGE_CURVE('',#43759,#43760,#23776,.T.);
#56011=EDGE_CURVE('',#43760,#43761,#2180,.T.);
#56012=EDGE_CURVE('',#43761,#43762,#23777,.T.);
#56013=EDGE_CURVE('',#43762,#43763,#2181,.T.);
#56014=EDGE_CURVE('',#43763,#43764,#23778,.T.);
#56015=EDGE_CURVE('',#43764,#43753,#23779,.T.);
#56016=EDGE_CURVE('',#43765,#43766,#23780,.T.);
#56017=EDGE_CURVE('',#43766,#43767,#34419,.T.);
#56018=EDGE_CURVE('',#43767,#43768,#23781,.T.);
#56019=EDGE_CURVE('',#43768,#43765,#34420,.T.);
#56020=EDGE_CURVE('',#43769,#43770,#2182,.T.);
#56021=EDGE_CURVE('',#43770,#43771,#23782,.T.);
#56022=EDGE_CURVE('',#43771,#43772,#23783,.T.);
#56023=EDGE_CURVE('',#43772,#43773,#23784,.T.);
#56024=EDGE_CURVE('',#43773,#43774,#2183,.T.);
#56025=EDGE_CURVE('',#43774,#43775,#23785,.T.);
#56026=EDGE_CURVE('',#43775,#43776,#23786,.T.);
#56027=EDGE_CURVE('',#43776,#43777,#2184,.T.);
#56028=EDGE_CURVE('',#43777,#43778,#23787,.T.);
#56029=EDGE_CURVE('',#43778,#43779,#2185,.T.);
#56030=EDGE_CURVE('',#43779,#43780,#23788,.T.);
#56031=EDGE_CURVE('',#43780,#43769,#23789,.T.);
#56032=EDGE_CURVE('',#43781,#43782,#2186,.T.);
#56033=EDGE_CURVE('',#43782,#43783,#23790,.T.);
#56034=EDGE_CURVE('',#43783,#43784,#23791,.T.);
#56035=EDGE_CURVE('',#43784,#43785,#23792,.T.);
#56036=EDGE_CURVE('',#43785,#43786,#2187,.T.);
#56037=EDGE_CURVE('',#43786,#43787,#23793,.T.);
#56038=EDGE_CURVE('',#43787,#43788,#23794,.T.);
#56039=EDGE_CURVE('',#43788,#43789,#2188,.T.);
#56040=EDGE_CURVE('',#43789,#43790,#23795,.T.);
#56041=EDGE_CURVE('',#43790,#43791,#2189,.T.);
#56042=EDGE_CURVE('',#43791,#43792,#23796,.T.);
#56043=EDGE_CURVE('',#43792,#43781,#23797,.T.);
#56044=EDGE_CURVE('',#43793,#43794,#23798,.T.);
#56045=EDGE_CURVE('',#43794,#43795,#34421,.T.);
#56046=EDGE_CURVE('',#43795,#43796,#23799,.T.);
#56047=EDGE_CURVE('',#43796,#43793,#34422,.T.);
#56048=EDGE_CURVE('',#43797,#43798,#2190,.T.);
#56049=EDGE_CURVE('',#43798,#43799,#23800,.T.);
#56050=EDGE_CURVE('',#43799,#43800,#23801,.T.);
#56051=EDGE_CURVE('',#43800,#43801,#23802,.T.);
#56052=EDGE_CURVE('',#43801,#43802,#2191,.T.);
#56053=EDGE_CURVE('',#43802,#43803,#23803,.T.);
#56054=EDGE_CURVE('',#43803,#43804,#23804,.T.);
#56055=EDGE_CURVE('',#43804,#43805,#2192,.T.);
#56056=EDGE_CURVE('',#43805,#43806,#23805,.T.);
#56057=EDGE_CURVE('',#43806,#43807,#2193,.T.);
#56058=EDGE_CURVE('',#43807,#43808,#23806,.T.);
#56059=EDGE_CURVE('',#43808,#43797,#23807,.T.);
#56060=EDGE_CURVE('',#43809,#43810,#2194,.T.);
#56061=EDGE_CURVE('',#43810,#43811,#23808,.T.);
#56062=EDGE_CURVE('',#43811,#43812,#23809,.T.);
#56063=EDGE_CURVE('',#43812,#43813,#23810,.T.);
#56064=EDGE_CURVE('',#43813,#43814,#2195,.T.);
#56065=EDGE_CURVE('',#43814,#43815,#23811,.T.);
#56066=EDGE_CURVE('',#43815,#43816,#23812,.T.);
#56067=EDGE_CURVE('',#43816,#43817,#2196,.T.);
#56068=EDGE_CURVE('',#43817,#43818,#23813,.T.);
#56069=EDGE_CURVE('',#43818,#43819,#2197,.T.);
#56070=EDGE_CURVE('',#43819,#43820,#23814,.T.);
#56071=EDGE_CURVE('',#43820,#43809,#23815,.T.);
#56072=EDGE_CURVE('',#43821,#43822,#23816,.T.);
#56073=EDGE_CURVE('',#43822,#43823,#34423,.T.);
#56074=EDGE_CURVE('',#43823,#43824,#23817,.T.);
#56075=EDGE_CURVE('',#43824,#43821,#34424,.T.);
#56076=EDGE_CURVE('',#43825,#43826,#2198,.T.);
#56077=EDGE_CURVE('',#43826,#43827,#23818,.T.);
#56078=EDGE_CURVE('',#43827,#43828,#23819,.T.);
#56079=EDGE_CURVE('',#43828,#43829,#23820,.T.);
#56080=EDGE_CURVE('',#43829,#43830,#2199,.T.);
#56081=EDGE_CURVE('',#43830,#43831,#23821,.T.);
#56082=EDGE_CURVE('',#43831,#43832,#23822,.T.);
#56083=EDGE_CURVE('',#43832,#43833,#2200,.T.);
#56084=EDGE_CURVE('',#43833,#43834,#23823,.T.);
#56085=EDGE_CURVE('',#43834,#43835,#2201,.T.);
#56086=EDGE_CURVE('',#43835,#43836,#23824,.T.);
#56087=EDGE_CURVE('',#43836,#43825,#23825,.T.);
#56088=EDGE_CURVE('',#43837,#43838,#2202,.T.);
#56089=EDGE_CURVE('',#43838,#43839,#23826,.T.);
#56090=EDGE_CURVE('',#43839,#43840,#23827,.T.);
#56091=EDGE_CURVE('',#43840,#43841,#23828,.T.);
#56092=EDGE_CURVE('',#43841,#43842,#2203,.T.);
#56093=EDGE_CURVE('',#43842,#43843,#23829,.T.);
#56094=EDGE_CURVE('',#43843,#43844,#23830,.T.);
#56095=EDGE_CURVE('',#43844,#43845,#2204,.T.);
#56096=EDGE_CURVE('',#43845,#43846,#23831,.T.);
#56097=EDGE_CURVE('',#43846,#43847,#2205,.T.);
#56098=EDGE_CURVE('',#43847,#43848,#23832,.T.);
#56099=EDGE_CURVE('',#43848,#43837,#23833,.T.);
#56100=EDGE_CURVE('',#43849,#43850,#23834,.T.);
#56101=EDGE_CURVE('',#43850,#43851,#34425,.T.);
#56102=EDGE_CURVE('',#43851,#43852,#23835,.T.);
#56103=EDGE_CURVE('',#43852,#43849,#34426,.T.);
#56104=EDGE_CURVE('',#43853,#43854,#2206,.T.);
#56105=EDGE_CURVE('',#43854,#43855,#23836,.T.);
#56106=EDGE_CURVE('',#43855,#43856,#23837,.T.);
#56107=EDGE_CURVE('',#43856,#43857,#23838,.T.);
#56108=EDGE_CURVE('',#43857,#43858,#2207,.T.);
#56109=EDGE_CURVE('',#43858,#43859,#23839,.T.);
#56110=EDGE_CURVE('',#43859,#43860,#23840,.T.);
#56111=EDGE_CURVE('',#43860,#43861,#2208,.T.);
#56112=EDGE_CURVE('',#43861,#43862,#23841,.T.);
#56113=EDGE_CURVE('',#43862,#43863,#2209,.T.);
#56114=EDGE_CURVE('',#43863,#43864,#23842,.T.);
#56115=EDGE_CURVE('',#43864,#43853,#23843,.T.);
#56116=EDGE_CURVE('',#43865,#43866,#2210,.T.);
#56117=EDGE_CURVE('',#43866,#43867,#23844,.T.);
#56118=EDGE_CURVE('',#43867,#43868,#23845,.T.);
#56119=EDGE_CURVE('',#43868,#43869,#23846,.T.);
#56120=EDGE_CURVE('',#43869,#43870,#2211,.T.);
#56121=EDGE_CURVE('',#43870,#43871,#23847,.T.);
#56122=EDGE_CURVE('',#43871,#43872,#23848,.T.);
#56123=EDGE_CURVE('',#43872,#43873,#2212,.T.);
#56124=EDGE_CURVE('',#43873,#43874,#23849,.T.);
#56125=EDGE_CURVE('',#43874,#43875,#2213,.T.);
#56126=EDGE_CURVE('',#43875,#43876,#23850,.T.);
#56127=EDGE_CURVE('',#43876,#43865,#23851,.T.);
#56128=EDGE_CURVE('',#43877,#43878,#23852,.T.);
#56129=EDGE_CURVE('',#43878,#43879,#34427,.T.);
#56130=EDGE_CURVE('',#43879,#43880,#23853,.T.);
#56131=EDGE_CURVE('',#43880,#43877,#34428,.T.);
#56132=EDGE_CURVE('',#43881,#43882,#2214,.T.);
#56133=EDGE_CURVE('',#43882,#43883,#23854,.T.);
#56134=EDGE_CURVE('',#43883,#43884,#23855,.T.);
#56135=EDGE_CURVE('',#43884,#43885,#23856,.T.);
#56136=EDGE_CURVE('',#43885,#43886,#2215,.T.);
#56137=EDGE_CURVE('',#43886,#43887,#23857,.T.);
#56138=EDGE_CURVE('',#43887,#43888,#23858,.T.);
#56139=EDGE_CURVE('',#43888,#43889,#2216,.T.);
#56140=EDGE_CURVE('',#43889,#43890,#23859,.T.);
#56141=EDGE_CURVE('',#43890,#43891,#2217,.T.);
#56142=EDGE_CURVE('',#43891,#43892,#23860,.T.);
#56143=EDGE_CURVE('',#43892,#43881,#23861,.T.);
#56144=EDGE_CURVE('',#43893,#43894,#2218,.T.);
#56145=EDGE_CURVE('',#43894,#43895,#23862,.T.);
#56146=EDGE_CURVE('',#43895,#43896,#23863,.T.);
#56147=EDGE_CURVE('',#43896,#43897,#23864,.T.);
#56148=EDGE_CURVE('',#43897,#43898,#2219,.T.);
#56149=EDGE_CURVE('',#43898,#43899,#23865,.T.);
#56150=EDGE_CURVE('',#43899,#43900,#23866,.T.);
#56151=EDGE_CURVE('',#43900,#43901,#2220,.T.);
#56152=EDGE_CURVE('',#43901,#43902,#23867,.T.);
#56153=EDGE_CURVE('',#43902,#43903,#2221,.T.);
#56154=EDGE_CURVE('',#43903,#43904,#23868,.T.);
#56155=EDGE_CURVE('',#43904,#43893,#23869,.T.);
#56156=EDGE_CURVE('',#43905,#43906,#23870,.T.);
#56157=EDGE_CURVE('',#43906,#43907,#34429,.T.);
#56158=EDGE_CURVE('',#43907,#43908,#23871,.T.);
#56159=EDGE_CURVE('',#43908,#43905,#34430,.T.);
#56160=EDGE_CURVE('',#43909,#43910,#2222,.T.);
#56161=EDGE_CURVE('',#43910,#43911,#23872,.T.);
#56162=EDGE_CURVE('',#43911,#43912,#23873,.T.);
#56163=EDGE_CURVE('',#43912,#43913,#23874,.T.);
#56164=EDGE_CURVE('',#43913,#43914,#2223,.T.);
#56165=EDGE_CURVE('',#43914,#43915,#23875,.T.);
#56166=EDGE_CURVE('',#43915,#43916,#23876,.T.);
#56167=EDGE_CURVE('',#43916,#43917,#2224,.T.);
#56168=EDGE_CURVE('',#43917,#43918,#23877,.T.);
#56169=EDGE_CURVE('',#43918,#43919,#2225,.T.);
#56170=EDGE_CURVE('',#43919,#43920,#23878,.T.);
#56171=EDGE_CURVE('',#43920,#43909,#23879,.T.);
#56172=EDGE_CURVE('',#43921,#43922,#2226,.T.);
#56173=EDGE_CURVE('',#43922,#43923,#23880,.T.);
#56174=EDGE_CURVE('',#43923,#43924,#23881,.T.);
#56175=EDGE_CURVE('',#43924,#43925,#23882,.T.);
#56176=EDGE_CURVE('',#43925,#43926,#2227,.T.);
#56177=EDGE_CURVE('',#43926,#43927,#23883,.T.);
#56178=EDGE_CURVE('',#43927,#43928,#23884,.T.);
#56179=EDGE_CURVE('',#43928,#43929,#2228,.T.);
#56180=EDGE_CURVE('',#43929,#43930,#23885,.T.);
#56181=EDGE_CURVE('',#43930,#43931,#2229,.T.);
#56182=EDGE_CURVE('',#43931,#43932,#23886,.T.);
#56183=EDGE_CURVE('',#43932,#43921,#23887,.T.);
#56184=EDGE_CURVE('',#43933,#43934,#23888,.T.);
#56185=EDGE_CURVE('',#43934,#43935,#34431,.T.);
#56186=EDGE_CURVE('',#43935,#43936,#23889,.T.);
#56187=EDGE_CURVE('',#43936,#43933,#34432,.T.);
#56188=EDGE_CURVE('',#43937,#43938,#2230,.T.);
#56189=EDGE_CURVE('',#43938,#43939,#23890,.T.);
#56190=EDGE_CURVE('',#43939,#43940,#23891,.T.);
#56191=EDGE_CURVE('',#43940,#43941,#23892,.T.);
#56192=EDGE_CURVE('',#43941,#43942,#2231,.T.);
#56193=EDGE_CURVE('',#43942,#43943,#23893,.T.);
#56194=EDGE_CURVE('',#43943,#43944,#23894,.T.);
#56195=EDGE_CURVE('',#43944,#43945,#2232,.T.);
#56196=EDGE_CURVE('',#43945,#43946,#23895,.T.);
#56197=EDGE_CURVE('',#43946,#43947,#2233,.T.);
#56198=EDGE_CURVE('',#43947,#43948,#23896,.T.);
#56199=EDGE_CURVE('',#43948,#43937,#23897,.T.);
#56200=EDGE_CURVE('',#43949,#43950,#2234,.T.);
#56201=EDGE_CURVE('',#43950,#43951,#23898,.T.);
#56202=EDGE_CURVE('',#43951,#43952,#23899,.T.);
#56203=EDGE_CURVE('',#43952,#43953,#23900,.T.);
#56204=EDGE_CURVE('',#43953,#43954,#2235,.T.);
#56205=EDGE_CURVE('',#43954,#43955,#23901,.T.);
#56206=EDGE_CURVE('',#43955,#43956,#23902,.T.);
#56207=EDGE_CURVE('',#43956,#43957,#2236,.T.);
#56208=EDGE_CURVE('',#43957,#43958,#23903,.T.);
#56209=EDGE_CURVE('',#43958,#43959,#2237,.T.);
#56210=EDGE_CURVE('',#43959,#43960,#23904,.T.);
#56211=EDGE_CURVE('',#43960,#43949,#23905,.T.);
#56212=EDGE_CURVE('',#43961,#43962,#23906,.T.);
#56213=EDGE_CURVE('',#43962,#43963,#34433,.T.);
#56214=EDGE_CURVE('',#43963,#43964,#23907,.T.);
#56215=EDGE_CURVE('',#43964,#43961,#34434,.T.);
#56216=EDGE_CURVE('',#43965,#43966,#2238,.T.);
#56217=EDGE_CURVE('',#43966,#43967,#23908,.T.);
#56218=EDGE_CURVE('',#43967,#43968,#23909,.T.);
#56219=EDGE_CURVE('',#43968,#43969,#23910,.T.);
#56220=EDGE_CURVE('',#43969,#43970,#2239,.T.);
#56221=EDGE_CURVE('',#43970,#43971,#23911,.T.);
#56222=EDGE_CURVE('',#43971,#43972,#23912,.T.);
#56223=EDGE_CURVE('',#43972,#43973,#2240,.T.);
#56224=EDGE_CURVE('',#43973,#43974,#23913,.T.);
#56225=EDGE_CURVE('',#43974,#43975,#2241,.T.);
#56226=EDGE_CURVE('',#43975,#43976,#23914,.T.);
#56227=EDGE_CURVE('',#43976,#43965,#23915,.T.);
#56228=EDGE_CURVE('',#43977,#43978,#2242,.T.);
#56229=EDGE_CURVE('',#43978,#43979,#23916,.T.);
#56230=EDGE_CURVE('',#43979,#43980,#23917,.T.);
#56231=EDGE_CURVE('',#43980,#43981,#23918,.T.);
#56232=EDGE_CURVE('',#43981,#43982,#2243,.T.);
#56233=EDGE_CURVE('',#43982,#43983,#23919,.T.);
#56234=EDGE_CURVE('',#43983,#43984,#23920,.T.);
#56235=EDGE_CURVE('',#43984,#43985,#2244,.T.);
#56236=EDGE_CURVE('',#43985,#43986,#23921,.T.);
#56237=EDGE_CURVE('',#43986,#43987,#2245,.T.);
#56238=EDGE_CURVE('',#43987,#43988,#23922,.T.);
#56239=EDGE_CURVE('',#43988,#43977,#23923,.T.);
#56240=EDGE_CURVE('',#43989,#43990,#23924,.T.);
#56241=EDGE_CURVE('',#43990,#43991,#34435,.T.);
#56242=EDGE_CURVE('',#43991,#43992,#23925,.T.);
#56243=EDGE_CURVE('',#43992,#43989,#34436,.T.);
#56244=EDGE_CURVE('',#43993,#43994,#2246,.T.);
#56245=EDGE_CURVE('',#43994,#43995,#23926,.T.);
#56246=EDGE_CURVE('',#43995,#43996,#23927,.T.);
#56247=EDGE_CURVE('',#43996,#43997,#23928,.T.);
#56248=EDGE_CURVE('',#43997,#43998,#2247,.T.);
#56249=EDGE_CURVE('',#43998,#43999,#23929,.T.);
#56250=EDGE_CURVE('',#43999,#44000,#23930,.T.);
#56251=EDGE_CURVE('',#44000,#44001,#2248,.T.);
#56252=EDGE_CURVE('',#44001,#44002,#23931,.T.);
#56253=EDGE_CURVE('',#44002,#44003,#2249,.T.);
#56254=EDGE_CURVE('',#44003,#44004,#23932,.T.);
#56255=EDGE_CURVE('',#44004,#43993,#23933,.T.);
#56256=EDGE_CURVE('',#44005,#44006,#2250,.T.);
#56257=EDGE_CURVE('',#44006,#44007,#23934,.T.);
#56258=EDGE_CURVE('',#44007,#44008,#23935,.T.);
#56259=EDGE_CURVE('',#44008,#44009,#23936,.T.);
#56260=EDGE_CURVE('',#44009,#44010,#2251,.T.);
#56261=EDGE_CURVE('',#44010,#44011,#23937,.T.);
#56262=EDGE_CURVE('',#44011,#44012,#23938,.T.);
#56263=EDGE_CURVE('',#44012,#44013,#2252,.T.);
#56264=EDGE_CURVE('',#44013,#44014,#23939,.T.);
#56265=EDGE_CURVE('',#44014,#44015,#2253,.T.);
#56266=EDGE_CURVE('',#44015,#44016,#23940,.T.);
#56267=EDGE_CURVE('',#44016,#44005,#23941,.T.);
#56268=EDGE_CURVE('',#44017,#44018,#23942,.T.);
#56269=EDGE_CURVE('',#44018,#44019,#34437,.T.);
#56270=EDGE_CURVE('',#44019,#44020,#23943,.T.);
#56271=EDGE_CURVE('',#44020,#44017,#34438,.T.);
#56272=EDGE_CURVE('',#44021,#44022,#2254,.T.);
#56273=EDGE_CURVE('',#44022,#44023,#23944,.T.);
#56274=EDGE_CURVE('',#44023,#44024,#23945,.T.);
#56275=EDGE_CURVE('',#44024,#44025,#23946,.T.);
#56276=EDGE_CURVE('',#44025,#44026,#2255,.T.);
#56277=EDGE_CURVE('',#44026,#44027,#23947,.T.);
#56278=EDGE_CURVE('',#44027,#44028,#23948,.T.);
#56279=EDGE_CURVE('',#44028,#44029,#2256,.T.);
#56280=EDGE_CURVE('',#44029,#44030,#23949,.T.);
#56281=EDGE_CURVE('',#44030,#44031,#2257,.T.);
#56282=EDGE_CURVE('',#44031,#44032,#23950,.T.);
#56283=EDGE_CURVE('',#44032,#44021,#23951,.T.);
#56284=EDGE_CURVE('',#44033,#44034,#2258,.T.);
#56285=EDGE_CURVE('',#44034,#44035,#23952,.T.);
#56286=EDGE_CURVE('',#44035,#44036,#23953,.T.);
#56287=EDGE_CURVE('',#44036,#44037,#23954,.T.);
#56288=EDGE_CURVE('',#44037,#44038,#2259,.T.);
#56289=EDGE_CURVE('',#44038,#44039,#23955,.T.);
#56290=EDGE_CURVE('',#44039,#44040,#23956,.T.);
#56291=EDGE_CURVE('',#44040,#44041,#2260,.T.);
#56292=EDGE_CURVE('',#44041,#44042,#23957,.T.);
#56293=EDGE_CURVE('',#44042,#44043,#2261,.T.);
#56294=EDGE_CURVE('',#44043,#44044,#23958,.T.);
#56295=EDGE_CURVE('',#44044,#44033,#23959,.T.);
#56296=EDGE_CURVE('',#42419,#42402,#4979,.T.);
#56297=EDGE_CURVE('',#42401,#42420,#4980,.T.);
#56298=EDGE_CURVE('',#42403,#42408,#4981,.T.);
#56299=EDGE_CURVE('',#42407,#42404,#4982,.T.);
#56300=EDGE_CURVE('',#42447,#42430,#4983,.T.);
#56301=EDGE_CURVE('',#42429,#42448,#4984,.T.);
#56302=EDGE_CURVE('',#42431,#42436,#4985,.T.);
#56303=EDGE_CURVE('',#42435,#42432,#4986,.T.);
#56304=EDGE_CURVE('',#42475,#42458,#4987,.T.);
#56305=EDGE_CURVE('',#42457,#42476,#4988,.T.);
#56306=EDGE_CURVE('',#42459,#42464,#4989,.T.);
#56307=EDGE_CURVE('',#42463,#42460,#4990,.T.);
#56308=EDGE_CURVE('',#42503,#42486,#4991,.T.);
#56309=EDGE_CURVE('',#42485,#42504,#4992,.T.);
#56310=EDGE_CURVE('',#42487,#42492,#4993,.T.);
#56311=EDGE_CURVE('',#42491,#42488,#4994,.T.);
#56312=EDGE_CURVE('',#42531,#42514,#4995,.T.);
#56313=EDGE_CURVE('',#42513,#42532,#4996,.T.);
#56314=EDGE_CURVE('',#42515,#42520,#4997,.T.);
#56315=EDGE_CURVE('',#42519,#42516,#4998,.T.);
#56316=EDGE_CURVE('',#42559,#42542,#4999,.T.);
#56317=EDGE_CURVE('',#42541,#42560,#5000,.T.);
#56318=EDGE_CURVE('',#42543,#42548,#5001,.T.);
#56319=EDGE_CURVE('',#42547,#42544,#5002,.T.);
#56320=EDGE_CURVE('',#42587,#42570,#5003,.T.);
#56321=EDGE_CURVE('',#42569,#42588,#5004,.T.);
#56322=EDGE_CURVE('',#42571,#42576,#5005,.T.);
#56323=EDGE_CURVE('',#42575,#42572,#5006,.T.);
#56324=EDGE_CURVE('',#42615,#42598,#5007,.T.);
#56325=EDGE_CURVE('',#42597,#42616,#5008,.T.);
#56326=EDGE_CURVE('',#42599,#42604,#5009,.T.);
#56327=EDGE_CURVE('',#42603,#42600,#5010,.T.);
#56328=EDGE_CURVE('',#42643,#42626,#5011,.T.);
#56329=EDGE_CURVE('',#42625,#42644,#5012,.T.);
#56330=EDGE_CURVE('',#42627,#42632,#5013,.T.);
#56331=EDGE_CURVE('',#42631,#42628,#5014,.T.);
#56332=EDGE_CURVE('',#42671,#42654,#5015,.T.);
#56333=EDGE_CURVE('',#42653,#42672,#5016,.T.);
#56334=EDGE_CURVE('',#42655,#42660,#5017,.T.);
#56335=EDGE_CURVE('',#42659,#42656,#5018,.T.);
#56336=EDGE_CURVE('',#42699,#42682,#5019,.T.);
#56337=EDGE_CURVE('',#42681,#42700,#5020,.T.);
#56338=EDGE_CURVE('',#42683,#42688,#5021,.T.);
#56339=EDGE_CURVE('',#42687,#42684,#5022,.T.);
#56340=EDGE_CURVE('',#42727,#42710,#5023,.T.);
#56341=EDGE_CURVE('',#42709,#42728,#5024,.T.);
#56342=EDGE_CURVE('',#42711,#42716,#5025,.T.);
#56343=EDGE_CURVE('',#42715,#42712,#5026,.T.);
#56344=EDGE_CURVE('',#42755,#42738,#5027,.T.);
#56345=EDGE_CURVE('',#42737,#42756,#5028,.T.);
#56346=EDGE_CURVE('',#42739,#42744,#5029,.T.);
#56347=EDGE_CURVE('',#42743,#42740,#5030,.T.);
#56348=EDGE_CURVE('',#42783,#42766,#5031,.T.);
#56349=EDGE_CURVE('',#42765,#42784,#5032,.T.);
#56350=EDGE_CURVE('',#42767,#42772,#5033,.T.);
#56351=EDGE_CURVE('',#42771,#42768,#5034,.T.);
#56352=EDGE_CURVE('',#42811,#42794,#5035,.T.);
#56353=EDGE_CURVE('',#42793,#42812,#5036,.T.);
#56354=EDGE_CURVE('',#42795,#42800,#5037,.T.);
#56355=EDGE_CURVE('',#42799,#42796,#5038,.T.);
#56356=EDGE_CURVE('',#42839,#42822,#5039,.T.);
#56357=EDGE_CURVE('',#42821,#42840,#5040,.T.);
#56358=EDGE_CURVE('',#42823,#42828,#5041,.T.);
#56359=EDGE_CURVE('',#42827,#42824,#5042,.T.);
#56360=EDGE_CURVE('',#42867,#42850,#5043,.T.);
#56361=EDGE_CURVE('',#42849,#42868,#5044,.T.);
#56362=EDGE_CURVE('',#42851,#42856,#5045,.T.);
#56363=EDGE_CURVE('',#42855,#42852,#5046,.T.);
#56364=EDGE_CURVE('',#42895,#42878,#5047,.T.);
#56365=EDGE_CURVE('',#42877,#42896,#5048,.T.);
#56366=EDGE_CURVE('',#42879,#42884,#5049,.T.);
#56367=EDGE_CURVE('',#42883,#42880,#5050,.T.);
#56368=EDGE_CURVE('',#42923,#42906,#5051,.T.);
#56369=EDGE_CURVE('',#42905,#42924,#5052,.T.);
#56370=EDGE_CURVE('',#42907,#42912,#5053,.T.);
#56371=EDGE_CURVE('',#42911,#42908,#5054,.T.);
#56372=EDGE_CURVE('',#42951,#42934,#5055,.T.);
#56373=EDGE_CURVE('',#42933,#42952,#5056,.T.);
#56374=EDGE_CURVE('',#42935,#42940,#5057,.T.);
#56375=EDGE_CURVE('',#42939,#42936,#5058,.T.);
#56376=EDGE_CURVE('',#42979,#42962,#5059,.T.);
#56377=EDGE_CURVE('',#42961,#42980,#5060,.T.);
#56378=EDGE_CURVE('',#42963,#42968,#5061,.T.);
#56379=EDGE_CURVE('',#42967,#42964,#5062,.T.);
#56380=EDGE_CURVE('',#43007,#42990,#5063,.T.);
#56381=EDGE_CURVE('',#42989,#43008,#5064,.T.);
#56382=EDGE_CURVE('',#42991,#42996,#5065,.T.);
#56383=EDGE_CURVE('',#42995,#42992,#5066,.T.);
#56384=EDGE_CURVE('',#43035,#43018,#5067,.T.);
#56385=EDGE_CURVE('',#43017,#43036,#5068,.T.);
#56386=EDGE_CURVE('',#43019,#43024,#5069,.T.);
#56387=EDGE_CURVE('',#43023,#43020,#5070,.T.);
#56388=EDGE_CURVE('',#43063,#43046,#5071,.T.);
#56389=EDGE_CURVE('',#43045,#43064,#5072,.T.);
#56390=EDGE_CURVE('',#43047,#43052,#5073,.T.);
#56391=EDGE_CURVE('',#43051,#43048,#5074,.T.);
#56392=EDGE_CURVE('',#43091,#43074,#5075,.T.);
#56393=EDGE_CURVE('',#43073,#43092,#5076,.T.);
#56394=EDGE_CURVE('',#43075,#43080,#5077,.T.);
#56395=EDGE_CURVE('',#43079,#43076,#5078,.T.);
#56396=EDGE_CURVE('',#43119,#43102,#5079,.T.);
#56397=EDGE_CURVE('',#43101,#43120,#5080,.T.);
#56398=EDGE_CURVE('',#43103,#43108,#5081,.T.);
#56399=EDGE_CURVE('',#43107,#43104,#5082,.T.);
#56400=EDGE_CURVE('',#43147,#43130,#5083,.T.);
#56401=EDGE_CURVE('',#43129,#43148,#5084,.T.);
#56402=EDGE_CURVE('',#43131,#43136,#5085,.T.);
#56403=EDGE_CURVE('',#43135,#43132,#5086,.T.);
#56404=EDGE_CURVE('',#43175,#43158,#5087,.T.);
#56405=EDGE_CURVE('',#43157,#43176,#5088,.T.);
#56406=EDGE_CURVE('',#43159,#43164,#5089,.T.);
#56407=EDGE_CURVE('',#43163,#43160,#5090,.T.);
#56408=EDGE_CURVE('',#43203,#43186,#5091,.T.);
#56409=EDGE_CURVE('',#43185,#43204,#5092,.T.);
#56410=EDGE_CURVE('',#43187,#43192,#5093,.T.);
#56411=EDGE_CURVE('',#43191,#43188,#5094,.T.);
#56412=EDGE_CURVE('',#43227,#40443,#5095,.T.);
#56413=EDGE_CURVE('',#40437,#43228,#5096,.T.);
#56414=EDGE_CURVE('',#40442,#43216,#5097,.T.);
#56415=EDGE_CURVE('',#43215,#40436,#5098,.T.);
#56416=EDGE_CURVE('',#43255,#43238,#5099,.T.);
#56417=EDGE_CURVE('',#43237,#43256,#5100,.T.);
#56418=EDGE_CURVE('',#43239,#43244,#5101,.T.);
#56419=EDGE_CURVE('',#43243,#43240,#5102,.T.);
#56420=EDGE_CURVE('',#43283,#43266,#5103,.T.);
#56421=EDGE_CURVE('',#43265,#43284,#5104,.T.);
#56422=EDGE_CURVE('',#43267,#43272,#5105,.T.);
#56423=EDGE_CURVE('',#43271,#43268,#5106,.T.);
#56424=EDGE_CURVE('',#43311,#43294,#5107,.T.);
#56425=EDGE_CURVE('',#43293,#43312,#5108,.T.);
#56426=EDGE_CURVE('',#43295,#43300,#5109,.T.);
#56427=EDGE_CURVE('',#43299,#43296,#5110,.T.);
#56428=EDGE_CURVE('',#43339,#43322,#5111,.T.);
#56429=EDGE_CURVE('',#43321,#43340,#5112,.T.);
#56430=EDGE_CURVE('',#43323,#43328,#5113,.T.);
#56431=EDGE_CURVE('',#43327,#43324,#5114,.T.);
#56432=EDGE_CURVE('',#43367,#43350,#5115,.T.);
#56433=EDGE_CURVE('',#43349,#43368,#5116,.T.);
#56434=EDGE_CURVE('',#43351,#43356,#5117,.T.);
#56435=EDGE_CURVE('',#43355,#43352,#5118,.T.);
#56436=EDGE_CURVE('',#43395,#43378,#5119,.T.);
#56437=EDGE_CURVE('',#43377,#43396,#5120,.T.);
#56438=EDGE_CURVE('',#43379,#43384,#5121,.T.);
#56439=EDGE_CURVE('',#43383,#43380,#5122,.T.);
#56440=EDGE_CURVE('',#43423,#43406,#5123,.T.);
#56441=EDGE_CURVE('',#43405,#43424,#5124,.T.);
#56442=EDGE_CURVE('',#43407,#43412,#5125,.T.);
#56443=EDGE_CURVE('',#43411,#43408,#5126,.T.);
#56444=EDGE_CURVE('',#43451,#43434,#5127,.T.);
#56445=EDGE_CURVE('',#43433,#43452,#5128,.T.);
#56446=EDGE_CURVE('',#43435,#43440,#5129,.T.);
#56447=EDGE_CURVE('',#43439,#43436,#5130,.T.);
#56448=EDGE_CURVE('',#43479,#43462,#5131,.T.);
#56449=EDGE_CURVE('',#43461,#43480,#5132,.T.);
#56450=EDGE_CURVE('',#43463,#43468,#5133,.T.);
#56451=EDGE_CURVE('',#43467,#43464,#5134,.T.);
#56452=EDGE_CURVE('',#43507,#43490,#5135,.T.);
#56453=EDGE_CURVE('',#43489,#43508,#5136,.T.);
#56454=EDGE_CURVE('',#43491,#43496,#5137,.T.);
#56455=EDGE_CURVE('',#43495,#43492,#5138,.T.);
#56456=EDGE_CURVE('',#43535,#43518,#5139,.T.);
#56457=EDGE_CURVE('',#43517,#43536,#5140,.T.);
#56458=EDGE_CURVE('',#43519,#43524,#5141,.T.);
#56459=EDGE_CURVE('',#43523,#43520,#5142,.T.);
#56460=EDGE_CURVE('',#43563,#43546,#5143,.T.);
#56461=EDGE_CURVE('',#43545,#43564,#5144,.T.);
#56462=EDGE_CURVE('',#43547,#43552,#5145,.T.);
#56463=EDGE_CURVE('',#43551,#43548,#5146,.T.);
#56464=EDGE_CURVE('',#43591,#43574,#5147,.T.);
#56465=EDGE_CURVE('',#43573,#43592,#5148,.T.);
#56466=EDGE_CURVE('',#43575,#43580,#5149,.T.);
#56467=EDGE_CURVE('',#43579,#43576,#5150,.T.);
#56468=EDGE_CURVE('',#43619,#43602,#5151,.T.);
#56469=EDGE_CURVE('',#43601,#43620,#5152,.T.);
#56470=EDGE_CURVE('',#43603,#43608,#5153,.T.);
#56471=EDGE_CURVE('',#43607,#43604,#5154,.T.);
#56472=EDGE_CURVE('',#43643,#40435,#5155,.T.);
#56473=EDGE_CURVE('',#40429,#43644,#5156,.T.);
#56474=EDGE_CURVE('',#40434,#43632,#5157,.T.);
#56475=EDGE_CURVE('',#43631,#40428,#5158,.T.);
#56476=EDGE_CURVE('',#43671,#43654,#5159,.T.);
#56477=EDGE_CURVE('',#43653,#43672,#5160,.T.);
#56478=EDGE_CURVE('',#43655,#43660,#5161,.T.);
#56479=EDGE_CURVE('',#43659,#43656,#5162,.T.);
#56480=EDGE_CURVE('',#43699,#43682,#5163,.T.);
#56481=EDGE_CURVE('',#43681,#43700,#5164,.T.);
#56482=EDGE_CURVE('',#43683,#43688,#5165,.T.);
#56483=EDGE_CURVE('',#43687,#43684,#5166,.T.);
#56484=EDGE_CURVE('',#43727,#43710,#5167,.T.);
#56485=EDGE_CURVE('',#43709,#43728,#5168,.T.);
#56486=EDGE_CURVE('',#43711,#43716,#5169,.T.);
#56487=EDGE_CURVE('',#43715,#43712,#5170,.T.);
#56488=EDGE_CURVE('',#43755,#43738,#5171,.T.);
#56489=EDGE_CURVE('',#43737,#43756,#5172,.T.);
#56490=EDGE_CURVE('',#43739,#43744,#5173,.T.);
#56491=EDGE_CURVE('',#43743,#43740,#5174,.T.);
#56492=EDGE_CURVE('',#43783,#43766,#5175,.T.);
#56493=EDGE_CURVE('',#43765,#43784,#5176,.T.);
#56494=EDGE_CURVE('',#43767,#43772,#5177,.T.);
#56495=EDGE_CURVE('',#43771,#43768,#5178,.T.);
#56496=EDGE_CURVE('',#43811,#43794,#5179,.T.);
#56497=EDGE_CURVE('',#43793,#43812,#5180,.T.);
#56498=EDGE_CURVE('',#43795,#43800,#5181,.T.);
#56499=EDGE_CURVE('',#43799,#43796,#5182,.T.);
#56500=EDGE_CURVE('',#43839,#43822,#5183,.T.);
#56501=EDGE_CURVE('',#43821,#43840,#5184,.T.);
#56502=EDGE_CURVE('',#43823,#43828,#5185,.T.);
#56503=EDGE_CURVE('',#43827,#43824,#5186,.T.);
#56504=EDGE_CURVE('',#43867,#43850,#5187,.T.);
#56505=EDGE_CURVE('',#43849,#43868,#5188,.T.);
#56506=EDGE_CURVE('',#43851,#43856,#5189,.T.);
#56507=EDGE_CURVE('',#43855,#43852,#5190,.T.);
#56508=EDGE_CURVE('',#43895,#43878,#5191,.T.);
#56509=EDGE_CURVE('',#43877,#43896,#5192,.T.);
#56510=EDGE_CURVE('',#43879,#43884,#5193,.T.);
#56511=EDGE_CURVE('',#43883,#43880,#5194,.T.);
#56512=EDGE_CURVE('',#43923,#43906,#5195,.T.);
#56513=EDGE_CURVE('',#43905,#43924,#5196,.T.);
#56514=EDGE_CURVE('',#43907,#43912,#5197,.T.);
#56515=EDGE_CURVE('',#43911,#43908,#5198,.T.);
#56516=EDGE_CURVE('',#43951,#43934,#5199,.T.);
#56517=EDGE_CURVE('',#43933,#43952,#5200,.T.);
#56518=EDGE_CURVE('',#43935,#43940,#5201,.T.);
#56519=EDGE_CURVE('',#43939,#43936,#5202,.T.);
#56520=EDGE_CURVE('',#43979,#43962,#5203,.T.);
#56521=EDGE_CURVE('',#43961,#43980,#5204,.T.);
#56522=EDGE_CURVE('',#43963,#43968,#5205,.T.);
#56523=EDGE_CURVE('',#43967,#43964,#5206,.T.);
#56524=EDGE_CURVE('',#44007,#43990,#5207,.T.);
#56525=EDGE_CURVE('',#43989,#44008,#5208,.T.);
#56526=EDGE_CURVE('',#43991,#43996,#5209,.T.);
#56527=EDGE_CURVE('',#43995,#43992,#5210,.T.);
#56528=EDGE_CURVE('',#44035,#44018,#5211,.T.);
#56529=EDGE_CURVE('',#44017,#44036,#5212,.T.);
#56530=EDGE_CURVE('',#44019,#44024,#5213,.T.);
#56531=EDGE_CURVE('',#44023,#44020,#5214,.T.);
#56532=EDGE_CURVE('',#42428,#42350,#2262,.T.);
#56533=EDGE_CURVE('',#42345,#42427,#34439,.T.);
#56534=EDGE_CURVE('',#42344,#42426,#34440,.T.);
#56535=EDGE_CURVE('',#42417,#42352,#34441,.T.);
#56536=EDGE_CURVE('',#42341,#42425,#34442,.T.);
#56537=EDGE_CURVE('',#42418,#40466,#34443,.T.);
#56538=EDGE_CURVE('',#42340,#42424,#34444,.T.);
#56539=EDGE_CURVE('',#42419,#40465,#34445,.T.);
#56540=EDGE_CURVE('',#42338,#42423,#2263,.T.);
#56541=EDGE_CURVE('',#42402,#40464,#34446,.T.);
#56542=EDGE_CURVE('',#42333,#42422,#34447,.T.);
#56543=EDGE_CURVE('',#42403,#40463,#34448,.T.);
#56544=EDGE_CURVE('',#40983,#42421,#34449,.T.);
#56545=EDGE_CURVE('',#42408,#40462,#34450,.T.);
#56546=EDGE_CURVE('',#40984,#42420,#34451,.T.);
#56547=EDGE_CURVE('',#42409,#40461,#34452,.T.);
#56548=EDGE_CURVE('',#40985,#42401,#34453,.T.);
#56549=EDGE_CURVE('',#42410,#42371,#34454,.T.);
#56550=EDGE_CURVE('',#40986,#42404,#34455,.T.);
#56551=EDGE_CURVE('',#42411,#42367,#2264,.T.);
#56552=EDGE_CURVE('',#40987,#42407,#34456,.T.);
#56553=EDGE_CURVE('',#42412,#42366,#34457,.T.);
#56554=EDGE_CURVE('',#40988,#42406,#34458,.T.);
#56555=EDGE_CURVE('',#42413,#42363,#34459,.T.);
#56556=EDGE_CURVE('',#42354,#42405,#34460,.T.);
#56557=EDGE_CURVE('',#42414,#42362,#34461,.T.);
#56558=EDGE_CURVE('',#42355,#42416,#2265,.T.);
#56559=EDGE_CURVE('',#42415,#42359,#34462,.T.);
#56560=EDGE_CURVE('',#42456,#42330,#2266,.T.);
#56561=EDGE_CURVE('',#42325,#42455,#34463,.T.);
#56562=EDGE_CURVE('',#42324,#42454,#34464,.T.);
#56563=EDGE_CURVE('',#42445,#42332,#34465,.T.);
#56564=EDGE_CURVE('',#42321,#42453,#34466,.T.);
#56565=EDGE_CURVE('',#42446,#40472,#34467,.T.);
#56566=EDGE_CURVE('',#42320,#42452,#34468,.T.);
#56567=EDGE_CURVE('',#42447,#40471,#34469,.T.);
#56568=EDGE_CURVE('',#42318,#42451,#2267,.T.);
#56569=EDGE_CURVE('',#42430,#40470,#34470,.T.);
#56570=EDGE_CURVE('',#42313,#42450,#34471,.T.);
#56571=EDGE_CURVE('',#42431,#40469,#34472,.T.);
#56572=EDGE_CURVE('',#40977,#42449,#34473,.T.);
#56573=EDGE_CURVE('',#42436,#40468,#34474,.T.);
#56574=EDGE_CURVE('',#40978,#42448,#34475,.T.);
#56575=EDGE_CURVE('',#42437,#40467,#34476,.T.);
#56576=EDGE_CURVE('',#40979,#42429,#34477,.T.);
#56577=EDGE_CURVE('',#42438,#42351,#34478,.T.);
#56578=EDGE_CURVE('',#40980,#42432,#34479,.T.);
#56579=EDGE_CURVE('',#42439,#42347,#2268,.T.);
#56580=EDGE_CURVE('',#40981,#42435,#34480,.T.);
#56581=EDGE_CURVE('',#42440,#42346,#34481,.T.);
#56582=EDGE_CURVE('',#40982,#42434,#34482,.T.);
#56583=EDGE_CURVE('',#42441,#42343,#34483,.T.);
#56584=EDGE_CURVE('',#42334,#42433,#34484,.T.);
#56585=EDGE_CURVE('',#42442,#42342,#34485,.T.);
#56586=EDGE_CURVE('',#42335,#42444,#2269,.T.);
#56587=EDGE_CURVE('',#42443,#42339,#34486,.T.);
#56588=EDGE_CURVE('',#42484,#42310,#2270,.T.);
#56589=EDGE_CURVE('',#42305,#42483,#34487,.T.);
#56590=EDGE_CURVE('',#42304,#42482,#34488,.T.);
#56591=EDGE_CURVE('',#42473,#42312,#34489,.T.);
#56592=EDGE_CURVE('',#42301,#42481,#34490,.T.);
#56593=EDGE_CURVE('',#42474,#40478,#34491,.T.);
#56594=EDGE_CURVE('',#42300,#42480,#34492,.T.);
#56595=EDGE_CURVE('',#42475,#40477,#34493,.T.);
#56596=EDGE_CURVE('',#42298,#42479,#2271,.T.);
#56597=EDGE_CURVE('',#42458,#40476,#34494,.T.);
#56598=EDGE_CURVE('',#42293,#42478,#34495,.T.);
#56599=EDGE_CURVE('',#42459,#40475,#34496,.T.);
#56600=EDGE_CURVE('',#40971,#42477,#34497,.T.);
#56601=EDGE_CURVE('',#42464,#40474,#34498,.T.);
#56602=EDGE_CURVE('',#40972,#42476,#34499,.T.);
#56603=EDGE_CURVE('',#42465,#40473,#34500,.T.);
#56604=EDGE_CURVE('',#40973,#42457,#34501,.T.);
#56605=EDGE_CURVE('',#42466,#42331,#34502,.T.);
#56606=EDGE_CURVE('',#40974,#42460,#34503,.T.);
#56607=EDGE_CURVE('',#42467,#42327,#2272,.T.);
#56608=EDGE_CURVE('',#40975,#42463,#34504,.T.);
#56609=EDGE_CURVE('',#42468,#42326,#34505,.T.);
#56610=EDGE_CURVE('',#40976,#42462,#34506,.T.);
#56611=EDGE_CURVE('',#42469,#42323,#34507,.T.);
#56612=EDGE_CURVE('',#42314,#42461,#34508,.T.);
#56613=EDGE_CURVE('',#42470,#42322,#34509,.T.);
#56614=EDGE_CURVE('',#42315,#42472,#2273,.T.);
#56615=EDGE_CURVE('',#42471,#42319,#34510,.T.);
#56616=EDGE_CURVE('',#42512,#42290,#2274,.T.);
#56617=EDGE_CURVE('',#42285,#42511,#34511,.T.);
#56618=EDGE_CURVE('',#42284,#42510,#34512,.T.);
#56619=EDGE_CURVE('',#42501,#42292,#34513,.T.);
#56620=EDGE_CURVE('',#42281,#42509,#34514,.T.);
#56621=EDGE_CURVE('',#42502,#40484,#34515,.T.);
#56622=EDGE_CURVE('',#42280,#42508,#34516,.T.);
#56623=EDGE_CURVE('',#42503,#40483,#34517,.T.);
#56624=EDGE_CURVE('',#42278,#42507,#2275,.T.);
#56625=EDGE_CURVE('',#42486,#40482,#34518,.T.);
#56626=EDGE_CURVE('',#42273,#42506,#34519,.T.);
#56627=EDGE_CURVE('',#42487,#40481,#34520,.T.);
#56628=EDGE_CURVE('',#40965,#42505,#34521,.T.);
#56629=EDGE_CURVE('',#42492,#40480,#34522,.T.);
#56630=EDGE_CURVE('',#40966,#42504,#34523,.T.);
#56631=EDGE_CURVE('',#42493,#40479,#34524,.T.);
#56632=EDGE_CURVE('',#40967,#42485,#34525,.T.);
#56633=EDGE_CURVE('',#42494,#42311,#34526,.T.);
#56634=EDGE_CURVE('',#40968,#42488,#34527,.T.);
#56635=EDGE_CURVE('',#42495,#42307,#2276,.T.);
#56636=EDGE_CURVE('',#40969,#42491,#34528,.T.);
#56637=EDGE_CURVE('',#42496,#42306,#34529,.T.);
#56638=EDGE_CURVE('',#40970,#42490,#34530,.T.);
#56639=EDGE_CURVE('',#42497,#42303,#34531,.T.);
#56640=EDGE_CURVE('',#42294,#42489,#34532,.T.);
#56641=EDGE_CURVE('',#42498,#42302,#34533,.T.);
#56642=EDGE_CURVE('',#42295,#42500,#2277,.T.);
#56643=EDGE_CURVE('',#42499,#42299,#34534,.T.);
#56644=EDGE_CURVE('',#42540,#42270,#2278,.T.);
#56645=EDGE_CURVE('',#42265,#42539,#34535,.T.);
#56646=EDGE_CURVE('',#42264,#42538,#34536,.T.);
#56647=EDGE_CURVE('',#42529,#42272,#34537,.T.);
#56648=EDGE_CURVE('',#42261,#42537,#34538,.T.);
#56649=EDGE_CURVE('',#42530,#40490,#34539,.T.);
#56650=EDGE_CURVE('',#42260,#42536,#34540,.T.);
#56651=EDGE_CURVE('',#42531,#40489,#34541,.T.);
#56652=EDGE_CURVE('',#42258,#42535,#2279,.T.);
#56653=EDGE_CURVE('',#42514,#40488,#34542,.T.);
#56654=EDGE_CURVE('',#42253,#42534,#34543,.T.);
#56655=EDGE_CURVE('',#42515,#40487,#34544,.T.);
#56656=EDGE_CURVE('',#40959,#42533,#34545,.T.);
#56657=EDGE_CURVE('',#42520,#40486,#34546,.T.);
#56658=EDGE_CURVE('',#40960,#42532,#34547,.T.);
#56659=EDGE_CURVE('',#42521,#40485,#34548,.T.);
#56660=EDGE_CURVE('',#40961,#42513,#34549,.T.);
#56661=EDGE_CURVE('',#42522,#42291,#34550,.T.);
#56662=EDGE_CURVE('',#40962,#42516,#34551,.T.);
#56663=EDGE_CURVE('',#42523,#42287,#2280,.T.);
#56664=EDGE_CURVE('',#40963,#42519,#34552,.T.);
#56665=EDGE_CURVE('',#42524,#42286,#34553,.T.);
#56666=EDGE_CURVE('',#40964,#42518,#34554,.T.);
#56667=EDGE_CURVE('',#42525,#42283,#34555,.T.);
#56668=EDGE_CURVE('',#42274,#42517,#34556,.T.);
#56669=EDGE_CURVE('',#42526,#42282,#34557,.T.);
#56670=EDGE_CURVE('',#42275,#42528,#2281,.T.);
#56671=EDGE_CURVE('',#42527,#42279,#34558,.T.);
#56672=EDGE_CURVE('',#42568,#42250,#2282,.T.);
#56673=EDGE_CURVE('',#42245,#42567,#34559,.T.);
#56674=EDGE_CURVE('',#42244,#42566,#34560,.T.);
#56675=EDGE_CURVE('',#42557,#42252,#34561,.T.);
#56676=EDGE_CURVE('',#42241,#42565,#34562,.T.);
#56677=EDGE_CURVE('',#42558,#40496,#34563,.T.);
#56678=EDGE_CURVE('',#42240,#42564,#34564,.T.);
#56679=EDGE_CURVE('',#42559,#40495,#34565,.T.);
#56680=EDGE_CURVE('',#42238,#42563,#2283,.T.);
#56681=EDGE_CURVE('',#42542,#40494,#34566,.T.);
#56682=EDGE_CURVE('',#42233,#42562,#34567,.T.);
#56683=EDGE_CURVE('',#42543,#40493,#34568,.T.);
#56684=EDGE_CURVE('',#40953,#42561,#34569,.T.);
#56685=EDGE_CURVE('',#42548,#40492,#34570,.T.);
#56686=EDGE_CURVE('',#40954,#42560,#34571,.T.);
#56687=EDGE_CURVE('',#42549,#40491,#34572,.T.);
#56688=EDGE_CURVE('',#40955,#42541,#34573,.T.);
#56689=EDGE_CURVE('',#42550,#42271,#34574,.T.);
#56690=EDGE_CURVE('',#40956,#42544,#34575,.T.);
#56691=EDGE_CURVE('',#42551,#42267,#2284,.T.);
#56692=EDGE_CURVE('',#40957,#42547,#34576,.T.);
#56693=EDGE_CURVE('',#42552,#42266,#34577,.T.);
#56694=EDGE_CURVE('',#40958,#42546,#34578,.T.);
#56695=EDGE_CURVE('',#42553,#42263,#34579,.T.);
#56696=EDGE_CURVE('',#42254,#42545,#34580,.T.);
#56697=EDGE_CURVE('',#42554,#42262,#34581,.T.);
#56698=EDGE_CURVE('',#42255,#42556,#2285,.T.);
#56699=EDGE_CURVE('',#42555,#42259,#34582,.T.);
#56700=EDGE_CURVE('',#42596,#42230,#2286,.T.);
#56701=EDGE_CURVE('',#42225,#42595,#34583,.T.);
#56702=EDGE_CURVE('',#42224,#42594,#34584,.T.);
#56703=EDGE_CURVE('',#42585,#42232,#34585,.T.);
#56704=EDGE_CURVE('',#42221,#42593,#34586,.T.);
#56705=EDGE_CURVE('',#42586,#40502,#34587,.T.);
#56706=EDGE_CURVE('',#42220,#42592,#34588,.T.);
#56707=EDGE_CURVE('',#42587,#40501,#34589,.T.);
#56708=EDGE_CURVE('',#42218,#42591,#2287,.T.);
#56709=EDGE_CURVE('',#42570,#40500,#34590,.T.);
#56710=EDGE_CURVE('',#42213,#42590,#34591,.T.);
#56711=EDGE_CURVE('',#42571,#40499,#34592,.T.);
#56712=EDGE_CURVE('',#40947,#42589,#34593,.T.);
#56713=EDGE_CURVE('',#42576,#40498,#34594,.T.);
#56714=EDGE_CURVE('',#40948,#42588,#34595,.T.);
#56715=EDGE_CURVE('',#42577,#40497,#34596,.T.);
#56716=EDGE_CURVE('',#40949,#42569,#34597,.T.);
#56717=EDGE_CURVE('',#42578,#42251,#34598,.T.);
#56718=EDGE_CURVE('',#40950,#42572,#34599,.T.);
#56719=EDGE_CURVE('',#42579,#42247,#2288,.T.);
#56720=EDGE_CURVE('',#40951,#42575,#34600,.T.);
#56721=EDGE_CURVE('',#42580,#42246,#34601,.T.);
#56722=EDGE_CURVE('',#40952,#42574,#34602,.T.);
#56723=EDGE_CURVE('',#42581,#42243,#34603,.T.);
#56724=EDGE_CURVE('',#42234,#42573,#34604,.T.);
#56725=EDGE_CURVE('',#42582,#42242,#34605,.T.);
#56726=EDGE_CURVE('',#42235,#42584,#2289,.T.);
#56727=EDGE_CURVE('',#42583,#42239,#34606,.T.);
#56728=EDGE_CURVE('',#42624,#42210,#2290,.T.);
#56729=EDGE_CURVE('',#42205,#42623,#34607,.T.);
#56730=EDGE_CURVE('',#42204,#42622,#34608,.T.);
#56731=EDGE_CURVE('',#42613,#42212,#34609,.T.);
#56732=EDGE_CURVE('',#42201,#42621,#34610,.T.);
#56733=EDGE_CURVE('',#42614,#40508,#34611,.T.);
#56734=EDGE_CURVE('',#42200,#42620,#34612,.T.);
#56735=EDGE_CURVE('',#42615,#40507,#34613,.T.);
#56736=EDGE_CURVE('',#42198,#42619,#2291,.T.);
#56737=EDGE_CURVE('',#42598,#40506,#34614,.T.);
#56738=EDGE_CURVE('',#42193,#42618,#34615,.T.);
#56739=EDGE_CURVE('',#42599,#40505,#34616,.T.);
#56740=EDGE_CURVE('',#40941,#42617,#34617,.T.);
#56741=EDGE_CURVE('',#42604,#40504,#34618,.T.);
#56742=EDGE_CURVE('',#40942,#42616,#34619,.T.);
#56743=EDGE_CURVE('',#42605,#40503,#34620,.T.);
#56744=EDGE_CURVE('',#40943,#42597,#34621,.T.);
#56745=EDGE_CURVE('',#42606,#42231,#34622,.T.);
#56746=EDGE_CURVE('',#40944,#42600,#34623,.T.);
#56747=EDGE_CURVE('',#42607,#42227,#2292,.T.);
#56748=EDGE_CURVE('',#40945,#42603,#34624,.T.);
#56749=EDGE_CURVE('',#42608,#42226,#34625,.T.);
#56750=EDGE_CURVE('',#40946,#42602,#34626,.T.);
#56751=EDGE_CURVE('',#42609,#42223,#34627,.T.);
#56752=EDGE_CURVE('',#42214,#42601,#34628,.T.);
#56753=EDGE_CURVE('',#42610,#42222,#34629,.T.);
#56754=EDGE_CURVE('',#42215,#42612,#2293,.T.);
#56755=EDGE_CURVE('',#42611,#42219,#34630,.T.);
#56756=EDGE_CURVE('',#42652,#42190,#2294,.T.);
#56757=EDGE_CURVE('',#42185,#42651,#34631,.T.);
#56758=EDGE_CURVE('',#42184,#42650,#34632,.T.);
#56759=EDGE_CURVE('',#42641,#42192,#34633,.T.);
#56760=EDGE_CURVE('',#42181,#42649,#34634,.T.);
#56761=EDGE_CURVE('',#42642,#40514,#34635,.T.);
#56762=EDGE_CURVE('',#42180,#42648,#34636,.T.);
#56763=EDGE_CURVE('',#42643,#40513,#34637,.T.);
#56764=EDGE_CURVE('',#42178,#42647,#2295,.T.);
#56765=EDGE_CURVE('',#42626,#40512,#34638,.T.);
#56766=EDGE_CURVE('',#42173,#42646,#34639,.T.);
#56767=EDGE_CURVE('',#42627,#40511,#34640,.T.);
#56768=EDGE_CURVE('',#40935,#42645,#34641,.T.);
#56769=EDGE_CURVE('',#42632,#40510,#34642,.T.);
#56770=EDGE_CURVE('',#40936,#42644,#34643,.T.);
#56771=EDGE_CURVE('',#42633,#40509,#34644,.T.);
#56772=EDGE_CURVE('',#40937,#42625,#34645,.T.);
#56773=EDGE_CURVE('',#42634,#42211,#34646,.T.);
#56774=EDGE_CURVE('',#40938,#42628,#34647,.T.);
#56775=EDGE_CURVE('',#42635,#42207,#2296,.T.);
#56776=EDGE_CURVE('',#40939,#42631,#34648,.T.);
#56777=EDGE_CURVE('',#42636,#42206,#34649,.T.);
#56778=EDGE_CURVE('',#40940,#42630,#34650,.T.);
#56779=EDGE_CURVE('',#42637,#42203,#34651,.T.);
#56780=EDGE_CURVE('',#42194,#42629,#34652,.T.);
#56781=EDGE_CURVE('',#42638,#42202,#34653,.T.);
#56782=EDGE_CURVE('',#42195,#42640,#2297,.T.);
#56783=EDGE_CURVE('',#42639,#42199,#34654,.T.);
#56784=EDGE_CURVE('',#42680,#42170,#2298,.T.);
#56785=EDGE_CURVE('',#42165,#42679,#34655,.T.);
#56786=EDGE_CURVE('',#42164,#42678,#34656,.T.);
#56787=EDGE_CURVE('',#42669,#42172,#34657,.T.);
#56788=EDGE_CURVE('',#42161,#42677,#34658,.T.);
#56789=EDGE_CURVE('',#42670,#40520,#34659,.T.);
#56790=EDGE_CURVE('',#42160,#42676,#34660,.T.);
#56791=EDGE_CURVE('',#42671,#40519,#34661,.T.);
#56792=EDGE_CURVE('',#42158,#42675,#2299,.T.);
#56793=EDGE_CURVE('',#42654,#40518,#34662,.T.);
#56794=EDGE_CURVE('',#42153,#42674,#34663,.T.);
#56795=EDGE_CURVE('',#42655,#40517,#34664,.T.);
#56796=EDGE_CURVE('',#40929,#42673,#34665,.T.);
#56797=EDGE_CURVE('',#42660,#40516,#34666,.T.);
#56798=EDGE_CURVE('',#40930,#42672,#34667,.T.);
#56799=EDGE_CURVE('',#42661,#40515,#34668,.T.);
#56800=EDGE_CURVE('',#40931,#42653,#34669,.T.);
#56801=EDGE_CURVE('',#42662,#42191,#34670,.T.);
#56802=EDGE_CURVE('',#40932,#42656,#34671,.T.);
#56803=EDGE_CURVE('',#42663,#42187,#2300,.T.);
#56804=EDGE_CURVE('',#40933,#42659,#34672,.T.);
#56805=EDGE_CURVE('',#42664,#42186,#34673,.T.);
#56806=EDGE_CURVE('',#40934,#42658,#34674,.T.);
#56807=EDGE_CURVE('',#42665,#42183,#34675,.T.);
#56808=EDGE_CURVE('',#42174,#42657,#34676,.T.);
#56809=EDGE_CURVE('',#42666,#42182,#34677,.T.);
#56810=EDGE_CURVE('',#42175,#42668,#2301,.T.);
#56811=EDGE_CURVE('',#42667,#42179,#34678,.T.);
#56812=EDGE_CURVE('',#42708,#42150,#2302,.T.);
#56813=EDGE_CURVE('',#42145,#42707,#34679,.T.);
#56814=EDGE_CURVE('',#42144,#42706,#34680,.T.);
#56815=EDGE_CURVE('',#42697,#42152,#34681,.T.);
#56816=EDGE_CURVE('',#42141,#42705,#34682,.T.);
#56817=EDGE_CURVE('',#42698,#40526,#34683,.T.);
#56818=EDGE_CURVE('',#42140,#42704,#34684,.T.);
#56819=EDGE_CURVE('',#42699,#40525,#34685,.T.);
#56820=EDGE_CURVE('',#42138,#42703,#2303,.T.);
#56821=EDGE_CURVE('',#42682,#40524,#34686,.T.);
#56822=EDGE_CURVE('',#42133,#42702,#34687,.T.);
#56823=EDGE_CURVE('',#42683,#40523,#34688,.T.);
#56824=EDGE_CURVE('',#40923,#42701,#34689,.T.);
#56825=EDGE_CURVE('',#42688,#40522,#34690,.T.);
#56826=EDGE_CURVE('',#40924,#42700,#34691,.T.);
#56827=EDGE_CURVE('',#42689,#40521,#34692,.T.);
#56828=EDGE_CURVE('',#40925,#42681,#34693,.T.);
#56829=EDGE_CURVE('',#42690,#42171,#34694,.T.);
#56830=EDGE_CURVE('',#40926,#42684,#34695,.T.);
#56831=EDGE_CURVE('',#42691,#42167,#2304,.T.);
#56832=EDGE_CURVE('',#40927,#42687,#34696,.T.);
#56833=EDGE_CURVE('',#42692,#42166,#34697,.T.);
#56834=EDGE_CURVE('',#40928,#42686,#34698,.T.);
#56835=EDGE_CURVE('',#42693,#42163,#34699,.T.);
#56836=EDGE_CURVE('',#42154,#42685,#34700,.T.);
#56837=EDGE_CURVE('',#42694,#42162,#34701,.T.);
#56838=EDGE_CURVE('',#42155,#42696,#2305,.T.);
#56839=EDGE_CURVE('',#42695,#42159,#34702,.T.);
#56840=EDGE_CURVE('',#42736,#42130,#2306,.T.);
#56841=EDGE_CURVE('',#42125,#42735,#34703,.T.);
#56842=EDGE_CURVE('',#42124,#42734,#34704,.T.);
#56843=EDGE_CURVE('',#42725,#42132,#34705,.T.);
#56844=EDGE_CURVE('',#42121,#42733,#34706,.T.);
#56845=EDGE_CURVE('',#42726,#40532,#34707,.T.);
#56846=EDGE_CURVE('',#42120,#42732,#34708,.T.);
#56847=EDGE_CURVE('',#42727,#40531,#34709,.T.);
#56848=EDGE_CURVE('',#42118,#42731,#2307,.T.);
#56849=EDGE_CURVE('',#42710,#40530,#34710,.T.);
#56850=EDGE_CURVE('',#42113,#42730,#34711,.T.);
#56851=EDGE_CURVE('',#42711,#40529,#34712,.T.);
#56852=EDGE_CURVE('',#40917,#42729,#34713,.T.);
#56853=EDGE_CURVE('',#42716,#40528,#34714,.T.);
#56854=EDGE_CURVE('',#40918,#42728,#34715,.T.);
#56855=EDGE_CURVE('',#42717,#40527,#34716,.T.);
#56856=EDGE_CURVE('',#40919,#42709,#34717,.T.);
#56857=EDGE_CURVE('',#42718,#42151,#34718,.T.);
#56858=EDGE_CURVE('',#40920,#42712,#34719,.T.);
#56859=EDGE_CURVE('',#42719,#42147,#2308,.T.);
#56860=EDGE_CURVE('',#40921,#42715,#34720,.T.);
#56861=EDGE_CURVE('',#42720,#42146,#34721,.T.);
#56862=EDGE_CURVE('',#40922,#42714,#34722,.T.);
#56863=EDGE_CURVE('',#42721,#42143,#34723,.T.);
#56864=EDGE_CURVE('',#42134,#42713,#34724,.T.);
#56865=EDGE_CURVE('',#42722,#42142,#34725,.T.);
#56866=EDGE_CURVE('',#42135,#42724,#2309,.T.);
#56867=EDGE_CURVE('',#42723,#42139,#34726,.T.);
#56868=EDGE_CURVE('',#42764,#42110,#2310,.T.);
#56869=EDGE_CURVE('',#42105,#42763,#34727,.T.);
#56870=EDGE_CURVE('',#42104,#42762,#34728,.T.);
#56871=EDGE_CURVE('',#42753,#42112,#34729,.T.);
#56872=EDGE_CURVE('',#42101,#42761,#34730,.T.);
#56873=EDGE_CURVE('',#42754,#40538,#34731,.T.);
#56874=EDGE_CURVE('',#42100,#42760,#34732,.T.);
#56875=EDGE_CURVE('',#42755,#40537,#34733,.T.);
#56876=EDGE_CURVE('',#42098,#42759,#2311,.T.);
#56877=EDGE_CURVE('',#42738,#40536,#34734,.T.);
#56878=EDGE_CURVE('',#42093,#42758,#34735,.T.);
#56879=EDGE_CURVE('',#42739,#40535,#34736,.T.);
#56880=EDGE_CURVE('',#40911,#42757,#34737,.T.);
#56881=EDGE_CURVE('',#42744,#40534,#34738,.T.);
#56882=EDGE_CURVE('',#40912,#42756,#34739,.T.);
#56883=EDGE_CURVE('',#42745,#40533,#34740,.T.);
#56884=EDGE_CURVE('',#40913,#42737,#34741,.T.);
#56885=EDGE_CURVE('',#42746,#42131,#34742,.T.);
#56886=EDGE_CURVE('',#40914,#42740,#34743,.T.);
#56887=EDGE_CURVE('',#42747,#42127,#2312,.T.);
#56888=EDGE_CURVE('',#40915,#42743,#34744,.T.);
#56889=EDGE_CURVE('',#42748,#42126,#34745,.T.);
#56890=EDGE_CURVE('',#40916,#42742,#34746,.T.);
#56891=EDGE_CURVE('',#42749,#42123,#34747,.T.);
#56892=EDGE_CURVE('',#42114,#42741,#34748,.T.);
#56893=EDGE_CURVE('',#42750,#42122,#34749,.T.);
#56894=EDGE_CURVE('',#42115,#42752,#2313,.T.);
#56895=EDGE_CURVE('',#42751,#42119,#34750,.T.);
#56896=EDGE_CURVE('',#42792,#42090,#2314,.T.);
#56897=EDGE_CURVE('',#42085,#42791,#34751,.T.);
#56898=EDGE_CURVE('',#42084,#42790,#34752,.T.);
#56899=EDGE_CURVE('',#42781,#42092,#34753,.T.);
#56900=EDGE_CURVE('',#42081,#42789,#34754,.T.);
#56901=EDGE_CURVE('',#42782,#40544,#34755,.T.);
#56902=EDGE_CURVE('',#42080,#42788,#34756,.T.);
#56903=EDGE_CURVE('',#42783,#40543,#34757,.T.);
#56904=EDGE_CURVE('',#42078,#42787,#2315,.T.);
#56905=EDGE_CURVE('',#42766,#40542,#34758,.T.);
#56906=EDGE_CURVE('',#42073,#42786,#34759,.T.);
#56907=EDGE_CURVE('',#42767,#40541,#34760,.T.);
#56908=EDGE_CURVE('',#40905,#42785,#34761,.T.);
#56909=EDGE_CURVE('',#42772,#40540,#34762,.T.);
#56910=EDGE_CURVE('',#40906,#42784,#34763,.T.);
#56911=EDGE_CURVE('',#42773,#40539,#34764,.T.);
#56912=EDGE_CURVE('',#40907,#42765,#34765,.T.);
#56913=EDGE_CURVE('',#42774,#42111,#34766,.T.);
#56914=EDGE_CURVE('',#40908,#42768,#34767,.T.);
#56915=EDGE_CURVE('',#42775,#42107,#2316,.T.);
#56916=EDGE_CURVE('',#40909,#42771,#34768,.T.);
#56917=EDGE_CURVE('',#42776,#42106,#34769,.T.);
#56918=EDGE_CURVE('',#40910,#42770,#34770,.T.);
#56919=EDGE_CURVE('',#42777,#42103,#34771,.T.);
#56920=EDGE_CURVE('',#42094,#42769,#34772,.T.);
#56921=EDGE_CURVE('',#42778,#42102,#34773,.T.);
#56922=EDGE_CURVE('',#42095,#42780,#2317,.T.);
#56923=EDGE_CURVE('',#42779,#42099,#34774,.T.);
#56924=EDGE_CURVE('',#42820,#42070,#2318,.T.);
#56925=EDGE_CURVE('',#42065,#42819,#34775,.T.);
#56926=EDGE_CURVE('',#42064,#42818,#34776,.T.);
#56927=EDGE_CURVE('',#42809,#42072,#34777,.T.);
#56928=EDGE_CURVE('',#42061,#42817,#34778,.T.);
#56929=EDGE_CURVE('',#42810,#40550,#34779,.T.);
#56930=EDGE_CURVE('',#42060,#42816,#34780,.T.);
#56931=EDGE_CURVE('',#42811,#40549,#34781,.T.);
#56932=EDGE_CURVE('',#42058,#42815,#2319,.T.);
#56933=EDGE_CURVE('',#42794,#40548,#34782,.T.);
#56934=EDGE_CURVE('',#42053,#42814,#34783,.T.);
#56935=EDGE_CURVE('',#42795,#40547,#34784,.T.);
#56936=EDGE_CURVE('',#40899,#42813,#34785,.T.);
#56937=EDGE_CURVE('',#42800,#40546,#34786,.T.);
#56938=EDGE_CURVE('',#40900,#42812,#34787,.T.);
#56939=EDGE_CURVE('',#42801,#40545,#34788,.T.);
#56940=EDGE_CURVE('',#40901,#42793,#34789,.T.);
#56941=EDGE_CURVE('',#42802,#42091,#34790,.T.);
#56942=EDGE_CURVE('',#40902,#42796,#34791,.T.);
#56943=EDGE_CURVE('',#42803,#42087,#2320,.T.);
#56944=EDGE_CURVE('',#40903,#42799,#34792,.T.);
#56945=EDGE_CURVE('',#42804,#42086,#34793,.T.);
#56946=EDGE_CURVE('',#40904,#42798,#34794,.T.);
#56947=EDGE_CURVE('',#42805,#42083,#34795,.T.);
#56948=EDGE_CURVE('',#42074,#42797,#34796,.T.);
#56949=EDGE_CURVE('',#42806,#42082,#34797,.T.);
#56950=EDGE_CURVE('',#42075,#42808,#2321,.T.);
#56951=EDGE_CURVE('',#42807,#42079,#34798,.T.);
#56952=EDGE_CURVE('',#42848,#42050,#2322,.T.);
#56953=EDGE_CURVE('',#42045,#42847,#34799,.T.);
#56954=EDGE_CURVE('',#42044,#42846,#34800,.T.);
#56955=EDGE_CURVE('',#42837,#42052,#34801,.T.);
#56956=EDGE_CURVE('',#42041,#42845,#34802,.T.);
#56957=EDGE_CURVE('',#42838,#40556,#34803,.T.);
#56958=EDGE_CURVE('',#42040,#42844,#34804,.T.);
#56959=EDGE_CURVE('',#42839,#40555,#34805,.T.);
#56960=EDGE_CURVE('',#42038,#42843,#2323,.T.);
#56961=EDGE_CURVE('',#42822,#40554,#34806,.T.);
#56962=EDGE_CURVE('',#42033,#42842,#34807,.T.);
#56963=EDGE_CURVE('',#42823,#40553,#34808,.T.);
#56964=EDGE_CURVE('',#40893,#42841,#34809,.T.);
#56965=EDGE_CURVE('',#42828,#40552,#34810,.T.);
#56966=EDGE_CURVE('',#40894,#42840,#34811,.T.);
#56967=EDGE_CURVE('',#42829,#40551,#34812,.T.);
#56968=EDGE_CURVE('',#40895,#42821,#34813,.T.);
#56969=EDGE_CURVE('',#42830,#42071,#34814,.T.);
#56970=EDGE_CURVE('',#40896,#42824,#34815,.T.);
#56971=EDGE_CURVE('',#42831,#42067,#2324,.T.);
#56972=EDGE_CURVE('',#40897,#42827,#34816,.T.);
#56973=EDGE_CURVE('',#42832,#42066,#34817,.T.);
#56974=EDGE_CURVE('',#40898,#42826,#34818,.T.);
#56975=EDGE_CURVE('',#42833,#42063,#34819,.T.);
#56976=EDGE_CURVE('',#42054,#42825,#34820,.T.);
#56977=EDGE_CURVE('',#42834,#42062,#34821,.T.);
#56978=EDGE_CURVE('',#42055,#42836,#2325,.T.);
#56979=EDGE_CURVE('',#42835,#42059,#34822,.T.);
#56980=EDGE_CURVE('',#42876,#42030,#2326,.T.);
#56981=EDGE_CURVE('',#42025,#42875,#34823,.T.);
#56982=EDGE_CURVE('',#42024,#42874,#34824,.T.);
#56983=EDGE_CURVE('',#42865,#42032,#34825,.T.);
#56984=EDGE_CURVE('',#42021,#42873,#34826,.T.);
#56985=EDGE_CURVE('',#42866,#40562,#34827,.T.);
#56986=EDGE_CURVE('',#42020,#42872,#34828,.T.);
#56987=EDGE_CURVE('',#42867,#40561,#34829,.T.);
#56988=EDGE_CURVE('',#42018,#42871,#2327,.T.);
#56989=EDGE_CURVE('',#42850,#40560,#34830,.T.);
#56990=EDGE_CURVE('',#42013,#42870,#34831,.T.);
#56991=EDGE_CURVE('',#42851,#40559,#34832,.T.);
#56992=EDGE_CURVE('',#40887,#42869,#34833,.T.);
#56993=EDGE_CURVE('',#42856,#40558,#34834,.T.);
#56994=EDGE_CURVE('',#40888,#42868,#34835,.T.);
#56995=EDGE_CURVE('',#42857,#40557,#34836,.T.);
#56996=EDGE_CURVE('',#40889,#42849,#34837,.T.);
#56997=EDGE_CURVE('',#42858,#42051,#34838,.T.);
#56998=EDGE_CURVE('',#40890,#42852,#34839,.T.);
#56999=EDGE_CURVE('',#42859,#42047,#2328,.T.);
#57000=EDGE_CURVE('',#40891,#42855,#34840,.T.);
#57001=EDGE_CURVE('',#42860,#42046,#34841,.T.);
#57002=EDGE_CURVE('',#40892,#42854,#34842,.T.);
#57003=EDGE_CURVE('',#42861,#42043,#34843,.T.);
#57004=EDGE_CURVE('',#42034,#42853,#34844,.T.);
#57005=EDGE_CURVE('',#42862,#42042,#34845,.T.);
#57006=EDGE_CURVE('',#42035,#42864,#2329,.T.);
#57007=EDGE_CURVE('',#42863,#42039,#34846,.T.);
#57008=EDGE_CURVE('',#42904,#42010,#2330,.T.);
#57009=EDGE_CURVE('',#42005,#42903,#34847,.T.);
#57010=EDGE_CURVE('',#42004,#42902,#34848,.T.);
#57011=EDGE_CURVE('',#42893,#42012,#34849,.T.);
#57012=EDGE_CURVE('',#42001,#42901,#34850,.T.);
#57013=EDGE_CURVE('',#42894,#40568,#34851,.T.);
#57014=EDGE_CURVE('',#42000,#42900,#34852,.T.);
#57015=EDGE_CURVE('',#42895,#40567,#34853,.T.);
#57016=EDGE_CURVE('',#41998,#42899,#2331,.T.);
#57017=EDGE_CURVE('',#42878,#40566,#34854,.T.);
#57018=EDGE_CURVE('',#41993,#42898,#34855,.T.);
#57019=EDGE_CURVE('',#42879,#40565,#34856,.T.);
#57020=EDGE_CURVE('',#40881,#42897,#34857,.T.);
#57021=EDGE_CURVE('',#42884,#40564,#34858,.T.);
#57022=EDGE_CURVE('',#40882,#42896,#34859,.T.);
#57023=EDGE_CURVE('',#42885,#40563,#34860,.T.);
#57024=EDGE_CURVE('',#40883,#42877,#34861,.T.);
#57025=EDGE_CURVE('',#42886,#42031,#34862,.T.);
#57026=EDGE_CURVE('',#40884,#42880,#34863,.T.);
#57027=EDGE_CURVE('',#42887,#42027,#2332,.T.);
#57028=EDGE_CURVE('',#40885,#42883,#34864,.T.);
#57029=EDGE_CURVE('',#42888,#42026,#34865,.T.);
#57030=EDGE_CURVE('',#40886,#42882,#34866,.T.);
#57031=EDGE_CURVE('',#42889,#42023,#34867,.T.);
#57032=EDGE_CURVE('',#42014,#42881,#34868,.T.);
#57033=EDGE_CURVE('',#42890,#42022,#34869,.T.);
#57034=EDGE_CURVE('',#42015,#42892,#2333,.T.);
#57035=EDGE_CURVE('',#42891,#42019,#34870,.T.);
#57036=EDGE_CURVE('',#42932,#41990,#2334,.T.);
#57037=EDGE_CURVE('',#41985,#42931,#34871,.T.);
#57038=EDGE_CURVE('',#41984,#42930,#34872,.T.);
#57039=EDGE_CURVE('',#42921,#41992,#34873,.T.);
#57040=EDGE_CURVE('',#41981,#42929,#34874,.T.);
#57041=EDGE_CURVE('',#42922,#40574,#34875,.T.);
#57042=EDGE_CURVE('',#41980,#42928,#34876,.T.);
#57043=EDGE_CURVE('',#42923,#40573,#34877,.T.);
#57044=EDGE_CURVE('',#41978,#42927,#2335,.T.);
#57045=EDGE_CURVE('',#42906,#40572,#34878,.T.);
#57046=EDGE_CURVE('',#41973,#42926,#34879,.T.);
#57047=EDGE_CURVE('',#42907,#40571,#34880,.T.);
#57048=EDGE_CURVE('',#40875,#42925,#34881,.T.);
#57049=EDGE_CURVE('',#42912,#40570,#34882,.T.);
#57050=EDGE_CURVE('',#40876,#42924,#34883,.T.);
#57051=EDGE_CURVE('',#42913,#40569,#34884,.T.);
#57052=EDGE_CURVE('',#40877,#42905,#34885,.T.);
#57053=EDGE_CURVE('',#42914,#42011,#34886,.T.);
#57054=EDGE_CURVE('',#40878,#42908,#34887,.T.);
#57055=EDGE_CURVE('',#42915,#42007,#2336,.T.);
#57056=EDGE_CURVE('',#40879,#42911,#34888,.T.);
#57057=EDGE_CURVE('',#42916,#42006,#34889,.T.);
#57058=EDGE_CURVE('',#40880,#42910,#34890,.T.);
#57059=EDGE_CURVE('',#42917,#42003,#34891,.T.);
#57060=EDGE_CURVE('',#41994,#42909,#34892,.T.);
#57061=EDGE_CURVE('',#42918,#42002,#34893,.T.);
#57062=EDGE_CURVE('',#41995,#42920,#2337,.T.);
#57063=EDGE_CURVE('',#42919,#41999,#34894,.T.);
#57064=EDGE_CURVE('',#42960,#41970,#2338,.T.);
#57065=EDGE_CURVE('',#41965,#42959,#34895,.T.);
#57066=EDGE_CURVE('',#41964,#42958,#34896,.T.);
#57067=EDGE_CURVE('',#42949,#41972,#34897,.T.);
#57068=EDGE_CURVE('',#41961,#42957,#34898,.T.);
#57069=EDGE_CURVE('',#42950,#40580,#34899,.T.);
#57070=EDGE_CURVE('',#41960,#42956,#34900,.T.);
#57071=EDGE_CURVE('',#42951,#40579,#34901,.T.);
#57072=EDGE_CURVE('',#41958,#42955,#2339,.T.);
#57073=EDGE_CURVE('',#42934,#40578,#34902,.T.);
#57074=EDGE_CURVE('',#41953,#42954,#34903,.T.);
#57075=EDGE_CURVE('',#42935,#40577,#34904,.T.);
#57076=EDGE_CURVE('',#40869,#42953,#34905,.T.);
#57077=EDGE_CURVE('',#42940,#40576,#34906,.T.);
#57078=EDGE_CURVE('',#40870,#42952,#34907,.T.);
#57079=EDGE_CURVE('',#42941,#40575,#34908,.T.);
#57080=EDGE_CURVE('',#40871,#42933,#34909,.T.);
#57081=EDGE_CURVE('',#42942,#41991,#34910,.T.);
#57082=EDGE_CURVE('',#40872,#42936,#34911,.T.);
#57083=EDGE_CURVE('',#42943,#41987,#2340,.T.);
#57084=EDGE_CURVE('',#40873,#42939,#34912,.T.);
#57085=EDGE_CURVE('',#42944,#41986,#34913,.T.);
#57086=EDGE_CURVE('',#40874,#42938,#34914,.T.);
#57087=EDGE_CURVE('',#42945,#41983,#34915,.T.);
#57088=EDGE_CURVE('',#41974,#42937,#34916,.T.);
#57089=EDGE_CURVE('',#42946,#41982,#34917,.T.);
#57090=EDGE_CURVE('',#41975,#42948,#2341,.T.);
#57091=EDGE_CURVE('',#42947,#41979,#34918,.T.);
#57092=EDGE_CURVE('',#42988,#41950,#2342,.T.);
#57093=EDGE_CURVE('',#41945,#42987,#34919,.T.);
#57094=EDGE_CURVE('',#41944,#42986,#34920,.T.);
#57095=EDGE_CURVE('',#42977,#41952,#34921,.T.);
#57096=EDGE_CURVE('',#41941,#42985,#34922,.T.);
#57097=EDGE_CURVE('',#42978,#40586,#34923,.T.);
#57098=EDGE_CURVE('',#41940,#42984,#34924,.T.);
#57099=EDGE_CURVE('',#42979,#40585,#34925,.T.);
#57100=EDGE_CURVE('',#41938,#42983,#2343,.T.);
#57101=EDGE_CURVE('',#42962,#40584,#34926,.T.);
#57102=EDGE_CURVE('',#41933,#42982,#34927,.T.);
#57103=EDGE_CURVE('',#42963,#40583,#34928,.T.);
#57104=EDGE_CURVE('',#40863,#42981,#34929,.T.);
#57105=EDGE_CURVE('',#42968,#40582,#34930,.T.);
#57106=EDGE_CURVE('',#40864,#42980,#34931,.T.);
#57107=EDGE_CURVE('',#42969,#40581,#34932,.T.);
#57108=EDGE_CURVE('',#40865,#42961,#34933,.T.);
#57109=EDGE_CURVE('',#42970,#41971,#34934,.T.);
#57110=EDGE_CURVE('',#40866,#42964,#34935,.T.);
#57111=EDGE_CURVE('',#42971,#41967,#2344,.T.);
#57112=EDGE_CURVE('',#40867,#42967,#34936,.T.);
#57113=EDGE_CURVE('',#42972,#41966,#34937,.T.);
#57114=EDGE_CURVE('',#40868,#42966,#34938,.T.);
#57115=EDGE_CURVE('',#42973,#41963,#34939,.T.);
#57116=EDGE_CURVE('',#41954,#42965,#34940,.T.);
#57117=EDGE_CURVE('',#42974,#41962,#34941,.T.);
#57118=EDGE_CURVE('',#41955,#42976,#2345,.T.);
#57119=EDGE_CURVE('',#42975,#41959,#34942,.T.);
#57120=EDGE_CURVE('',#43016,#41930,#2346,.T.);
#57121=EDGE_CURVE('',#41925,#43015,#34943,.T.);
#57122=EDGE_CURVE('',#41924,#43014,#34944,.T.);
#57123=EDGE_CURVE('',#43005,#41932,#34945,.T.);
#57124=EDGE_CURVE('',#41921,#43013,#34946,.T.);
#57125=EDGE_CURVE('',#43006,#40592,#34947,.T.);
#57126=EDGE_CURVE('',#41920,#43012,#34948,.T.);
#57127=EDGE_CURVE('',#43007,#40591,#34949,.T.);
#57128=EDGE_CURVE('',#41918,#43011,#2347,.T.);
#57129=EDGE_CURVE('',#42990,#40590,#34950,.T.);
#57130=EDGE_CURVE('',#41913,#43010,#34951,.T.);
#57131=EDGE_CURVE('',#42991,#40589,#34952,.T.);
#57132=EDGE_CURVE('',#40857,#43009,#34953,.T.);
#57133=EDGE_CURVE('',#42996,#40588,#34954,.T.);
#57134=EDGE_CURVE('',#40858,#43008,#34955,.T.);
#57135=EDGE_CURVE('',#42997,#40587,#34956,.T.);
#57136=EDGE_CURVE('',#40859,#42989,#34957,.T.);
#57137=EDGE_CURVE('',#42998,#41951,#34958,.T.);
#57138=EDGE_CURVE('',#40860,#42992,#34959,.T.);
#57139=EDGE_CURVE('',#42999,#41947,#2348,.T.);
#57140=EDGE_CURVE('',#40861,#42995,#34960,.T.);
#57141=EDGE_CURVE('',#43000,#41946,#34961,.T.);
#57142=EDGE_CURVE('',#40862,#42994,#34962,.T.);
#57143=EDGE_CURVE('',#43001,#41943,#34963,.T.);
#57144=EDGE_CURVE('',#41934,#42993,#34964,.T.);
#57145=EDGE_CURVE('',#43002,#41942,#34965,.T.);
#57146=EDGE_CURVE('',#41935,#43004,#2349,.T.);
#57147=EDGE_CURVE('',#43003,#41939,#34966,.T.);
#57148=EDGE_CURVE('',#43044,#41910,#2350,.T.);
#57149=EDGE_CURVE('',#41905,#43043,#34967,.T.);
#57150=EDGE_CURVE('',#41904,#43042,#34968,.T.);
#57151=EDGE_CURVE('',#43033,#41912,#34969,.T.);
#57152=EDGE_CURVE('',#41901,#43041,#34970,.T.);
#57153=EDGE_CURVE('',#43034,#40598,#34971,.T.);
#57154=EDGE_CURVE('',#41900,#43040,#34972,.T.);
#57155=EDGE_CURVE('',#43035,#40597,#34973,.T.);
#57156=EDGE_CURVE('',#41898,#43039,#2351,.T.);
#57157=EDGE_CURVE('',#43018,#40596,#34974,.T.);
#57158=EDGE_CURVE('',#41893,#43038,#34975,.T.);
#57159=EDGE_CURVE('',#43019,#40595,#34976,.T.);
#57160=EDGE_CURVE('',#40851,#43037,#34977,.T.);
#57161=EDGE_CURVE('',#43024,#40594,#34978,.T.);
#57162=EDGE_CURVE('',#40852,#43036,#34979,.T.);
#57163=EDGE_CURVE('',#43025,#40593,#34980,.T.);
#57164=EDGE_CURVE('',#40853,#43017,#34981,.T.);
#57165=EDGE_CURVE('',#43026,#41931,#34982,.T.);
#57166=EDGE_CURVE('',#40854,#43020,#34983,.T.);
#57167=EDGE_CURVE('',#43027,#41927,#2352,.T.);
#57168=EDGE_CURVE('',#40855,#43023,#34984,.T.);
#57169=EDGE_CURVE('',#43028,#41926,#34985,.T.);
#57170=EDGE_CURVE('',#40856,#43022,#34986,.T.);
#57171=EDGE_CURVE('',#43029,#41923,#34987,.T.);
#57172=EDGE_CURVE('',#41914,#43021,#34988,.T.);
#57173=EDGE_CURVE('',#43030,#41922,#34989,.T.);
#57174=EDGE_CURVE('',#41915,#43032,#2353,.T.);
#57175=EDGE_CURVE('',#43031,#41919,#34990,.T.);
#57176=EDGE_CURVE('',#43072,#41890,#2354,.T.);
#57177=EDGE_CURVE('',#41885,#43071,#34991,.T.);
#57178=EDGE_CURVE('',#41884,#43070,#34992,.T.);
#57179=EDGE_CURVE('',#43061,#41892,#34993,.T.);
#57180=EDGE_CURVE('',#41881,#43069,#34994,.T.);
#57181=EDGE_CURVE('',#43062,#40604,#34995,.T.);
#57182=EDGE_CURVE('',#41880,#43068,#34996,.T.);
#57183=EDGE_CURVE('',#43063,#40603,#34997,.T.);
#57184=EDGE_CURVE('',#41878,#43067,#2355,.T.);
#57185=EDGE_CURVE('',#43046,#40602,#34998,.T.);
#57186=EDGE_CURVE('',#41873,#43066,#34999,.T.);
#57187=EDGE_CURVE('',#43047,#40601,#35000,.T.);
#57188=EDGE_CURVE('',#40845,#43065,#35001,.T.);
#57189=EDGE_CURVE('',#43052,#40600,#35002,.T.);
#57190=EDGE_CURVE('',#40846,#43064,#35003,.T.);
#57191=EDGE_CURVE('',#43053,#40599,#35004,.T.);
#57192=EDGE_CURVE('',#40847,#43045,#35005,.T.);
#57193=EDGE_CURVE('',#43054,#41911,#35006,.T.);
#57194=EDGE_CURVE('',#40848,#43048,#35007,.T.);
#57195=EDGE_CURVE('',#43055,#41907,#2356,.T.);
#57196=EDGE_CURVE('',#40849,#43051,#35008,.T.);
#57197=EDGE_CURVE('',#43056,#41906,#35009,.T.);
#57198=EDGE_CURVE('',#40850,#43050,#35010,.T.);
#57199=EDGE_CURVE('',#43057,#41903,#35011,.T.);
#57200=EDGE_CURVE('',#41894,#43049,#35012,.T.);
#57201=EDGE_CURVE('',#43058,#41902,#35013,.T.);
#57202=EDGE_CURVE('',#41895,#43060,#2357,.T.);
#57203=EDGE_CURVE('',#43059,#41899,#35014,.T.);
#57204=EDGE_CURVE('',#43100,#41870,#2358,.T.);
#57205=EDGE_CURVE('',#41865,#43099,#35015,.T.);
#57206=EDGE_CURVE('',#41864,#43098,#35016,.T.);
#57207=EDGE_CURVE('',#43089,#41872,#35017,.T.);
#57208=EDGE_CURVE('',#41861,#43097,#35018,.T.);
#57209=EDGE_CURVE('',#43090,#40610,#35019,.T.);
#57210=EDGE_CURVE('',#41860,#43096,#35020,.T.);
#57211=EDGE_CURVE('',#43091,#40609,#35021,.T.);
#57212=EDGE_CURVE('',#41858,#43095,#2359,.T.);
#57213=EDGE_CURVE('',#43074,#40608,#35022,.T.);
#57214=EDGE_CURVE('',#41853,#43094,#35023,.T.);
#57215=EDGE_CURVE('',#43075,#40607,#35024,.T.);
#57216=EDGE_CURVE('',#40839,#43093,#35025,.T.);
#57217=EDGE_CURVE('',#43080,#40606,#35026,.T.);
#57218=EDGE_CURVE('',#40840,#43092,#35027,.T.);
#57219=EDGE_CURVE('',#43081,#40605,#35028,.T.);
#57220=EDGE_CURVE('',#40841,#43073,#35029,.T.);
#57221=EDGE_CURVE('',#43082,#41891,#35030,.T.);
#57222=EDGE_CURVE('',#40842,#43076,#35031,.T.);
#57223=EDGE_CURVE('',#43083,#41887,#2360,.T.);
#57224=EDGE_CURVE('',#40843,#43079,#35032,.T.);
#57225=EDGE_CURVE('',#43084,#41886,#35033,.T.);
#57226=EDGE_CURVE('',#40844,#43078,#35034,.T.);
#57227=EDGE_CURVE('',#43085,#41883,#35035,.T.);
#57228=EDGE_CURVE('',#41874,#43077,#35036,.T.);
#57229=EDGE_CURVE('',#43086,#41882,#35037,.T.);
#57230=EDGE_CURVE('',#41875,#43088,#2361,.T.);
#57231=EDGE_CURVE('',#43087,#41879,#35038,.T.);
#57232=EDGE_CURVE('',#43128,#41850,#2362,.T.);
#57233=EDGE_CURVE('',#41845,#43127,#35039,.T.);
#57234=EDGE_CURVE('',#41844,#43126,#35040,.T.);
#57235=EDGE_CURVE('',#43117,#41852,#35041,.T.);
#57236=EDGE_CURVE('',#41841,#43125,#35042,.T.);
#57237=EDGE_CURVE('',#43118,#40616,#35043,.T.);
#57238=EDGE_CURVE('',#41840,#43124,#35044,.T.);
#57239=EDGE_CURVE('',#43119,#40615,#35045,.T.);
#57240=EDGE_CURVE('',#41838,#43123,#2363,.T.);
#57241=EDGE_CURVE('',#43102,#40614,#35046,.T.);
#57242=EDGE_CURVE('',#41833,#43122,#35047,.T.);
#57243=EDGE_CURVE('',#43103,#40613,#35048,.T.);
#57244=EDGE_CURVE('',#40833,#43121,#35049,.T.);
#57245=EDGE_CURVE('',#43108,#40612,#35050,.T.);
#57246=EDGE_CURVE('',#40834,#43120,#35051,.T.);
#57247=EDGE_CURVE('',#43109,#40611,#35052,.T.);
#57248=EDGE_CURVE('',#40835,#43101,#35053,.T.);
#57249=EDGE_CURVE('',#43110,#41871,#35054,.T.);
#57250=EDGE_CURVE('',#40836,#43104,#35055,.T.);
#57251=EDGE_CURVE('',#43111,#41867,#2364,.T.);
#57252=EDGE_CURVE('',#40837,#43107,#35056,.T.);
#57253=EDGE_CURVE('',#43112,#41866,#35057,.T.);
#57254=EDGE_CURVE('',#40838,#43106,#35058,.T.);
#57255=EDGE_CURVE('',#43113,#41863,#35059,.T.);
#57256=EDGE_CURVE('',#41854,#43105,#35060,.T.);
#57257=EDGE_CURVE('',#43114,#41862,#35061,.T.);
#57258=EDGE_CURVE('',#41855,#43116,#2365,.T.);
#57259=EDGE_CURVE('',#43115,#41859,#35062,.T.);
#57260=EDGE_CURVE('',#43156,#41830,#2366,.T.);
#57261=EDGE_CURVE('',#41825,#43155,#35063,.T.);
#57262=EDGE_CURVE('',#41824,#43154,#35064,.T.);
#57263=EDGE_CURVE('',#43145,#41832,#35065,.T.);
#57264=EDGE_CURVE('',#41821,#43153,#35066,.T.);
#57265=EDGE_CURVE('',#43146,#40622,#35067,.T.);
#57266=EDGE_CURVE('',#41820,#43152,#35068,.T.);
#57267=EDGE_CURVE('',#43147,#40621,#35069,.T.);
#57268=EDGE_CURVE('',#41818,#43151,#2367,.T.);
#57269=EDGE_CURVE('',#43130,#40620,#35070,.T.);
#57270=EDGE_CURVE('',#41813,#43150,#35071,.T.);
#57271=EDGE_CURVE('',#43131,#40619,#35072,.T.);
#57272=EDGE_CURVE('',#40827,#43149,#35073,.T.);
#57273=EDGE_CURVE('',#43136,#40618,#35074,.T.);
#57274=EDGE_CURVE('',#40828,#43148,#35075,.T.);
#57275=EDGE_CURVE('',#43137,#40617,#35076,.T.);
#57276=EDGE_CURVE('',#40829,#43129,#35077,.T.);
#57277=EDGE_CURVE('',#43138,#41851,#35078,.T.);
#57278=EDGE_CURVE('',#40830,#43132,#35079,.T.);
#57279=EDGE_CURVE('',#43139,#41847,#2368,.T.);
#57280=EDGE_CURVE('',#40831,#43135,#35080,.T.);
#57281=EDGE_CURVE('',#43140,#41846,#35081,.T.);
#57282=EDGE_CURVE('',#40832,#43134,#35082,.T.);
#57283=EDGE_CURVE('',#43141,#41843,#35083,.T.);
#57284=EDGE_CURVE('',#41834,#43133,#35084,.T.);
#57285=EDGE_CURVE('',#43142,#41842,#35085,.T.);
#57286=EDGE_CURVE('',#41835,#43144,#2369,.T.);
#57287=EDGE_CURVE('',#43143,#41839,#35086,.T.);
#57288=EDGE_CURVE('',#43184,#41810,#2370,.T.);
#57289=EDGE_CURVE('',#41805,#43183,#35087,.T.);
#57290=EDGE_CURVE('',#41804,#43182,#35088,.T.);
#57291=EDGE_CURVE('',#43173,#41812,#35089,.T.);
#57292=EDGE_CURVE('',#41801,#43181,#35090,.T.);
#57293=EDGE_CURVE('',#43174,#40628,#35091,.T.);
#57294=EDGE_CURVE('',#41800,#43180,#35092,.T.);
#57295=EDGE_CURVE('',#43175,#40627,#35093,.T.);
#57296=EDGE_CURVE('',#41798,#43179,#2371,.T.);
#57297=EDGE_CURVE('',#43158,#40626,#35094,.T.);
#57298=EDGE_CURVE('',#41793,#43178,#35095,.T.);
#57299=EDGE_CURVE('',#43159,#40625,#35096,.T.);
#57300=EDGE_CURVE('',#40821,#43177,#35097,.T.);
#57301=EDGE_CURVE('',#43164,#40624,#35098,.T.);
#57302=EDGE_CURVE('',#40822,#43176,#35099,.T.);
#57303=EDGE_CURVE('',#43165,#40623,#35100,.T.);
#57304=EDGE_CURVE('',#40823,#43157,#35101,.T.);
#57305=EDGE_CURVE('',#43166,#41831,#35102,.T.);
#57306=EDGE_CURVE('',#40824,#43160,#35103,.T.);
#57307=EDGE_CURVE('',#43167,#41827,#2372,.T.);
#57308=EDGE_CURVE('',#40825,#43163,#35104,.T.);
#57309=EDGE_CURVE('',#43168,#41826,#35105,.T.);
#57310=EDGE_CURVE('',#40826,#43162,#35106,.T.);
#57311=EDGE_CURVE('',#43169,#41823,#35107,.T.);
#57312=EDGE_CURVE('',#41814,#43161,#35108,.T.);
#57313=EDGE_CURVE('',#43170,#41822,#35109,.T.);
#57314=EDGE_CURVE('',#41815,#43172,#2373,.T.);
#57315=EDGE_CURVE('',#43171,#41819,#35110,.T.);
#57316=EDGE_CURVE('',#43212,#41790,#2374,.T.);
#57317=EDGE_CURVE('',#41785,#43211,#35111,.T.);
#57318=EDGE_CURVE('',#41784,#43210,#35112,.T.);
#57319=EDGE_CURVE('',#43201,#41792,#35113,.T.);
#57320=EDGE_CURVE('',#41781,#43209,#35114,.T.);
#57321=EDGE_CURVE('',#43202,#40634,#35115,.T.);
#57322=EDGE_CURVE('',#41780,#43208,#35116,.T.);
#57323=EDGE_CURVE('',#43203,#40633,#35117,.T.);
#57324=EDGE_CURVE('',#41778,#43207,#2375,.T.);
#57325=EDGE_CURVE('',#43186,#40632,#35118,.T.);
#57326=EDGE_CURVE('',#41773,#43206,#35119,.T.);
#57327=EDGE_CURVE('',#43187,#40631,#35120,.T.);
#57328=EDGE_CURVE('',#40815,#43205,#35121,.T.);
#57329=EDGE_CURVE('',#43192,#40630,#35122,.T.);
#57330=EDGE_CURVE('',#40816,#43204,#35123,.T.);
#57331=EDGE_CURVE('',#43193,#40629,#35124,.T.);
#57332=EDGE_CURVE('',#40817,#43185,#35125,.T.);
#57333=EDGE_CURVE('',#43194,#41811,#35126,.T.);
#57334=EDGE_CURVE('',#40818,#43188,#35127,.T.);
#57335=EDGE_CURVE('',#43195,#41807,#2376,.T.);
#57336=EDGE_CURVE('',#40819,#43191,#35128,.T.);
#57337=EDGE_CURVE('',#43196,#41806,#35129,.T.);
#57338=EDGE_CURVE('',#40820,#43190,#35130,.T.);
#57339=EDGE_CURVE('',#43197,#41803,#35131,.T.);
#57340=EDGE_CURVE('',#41794,#43189,#35132,.T.);
#57341=EDGE_CURVE('',#43198,#41802,#35133,.T.);
#57342=EDGE_CURVE('',#41795,#43200,#2377,.T.);
#57343=EDGE_CURVE('',#43199,#41799,#35134,.T.);
#57344=EDGE_CURVE('',#43236,#41770,#2378,.T.);
#57345=EDGE_CURVE('',#41765,#43235,#35135,.T.);
#57346=EDGE_CURVE('',#41764,#43234,#35136,.T.);
#57347=EDGE_CURVE('',#43225,#41772,#35137,.T.);
#57348=EDGE_CURVE('',#41761,#43233,#35138,.T.);
#57349=EDGE_CURVE('',#43226,#40638,#35139,.T.);
#57350=EDGE_CURVE('',#41760,#43232,#35140,.T.);
#57351=EDGE_CURVE('',#43227,#40637,#35141,.T.);
#57352=EDGE_CURVE('',#41758,#43231,#2379,.T.);
#57353=EDGE_CURVE('',#41753,#43230,#35142,.T.);
#57354=EDGE_CURVE('',#41168,#43229,#35143,.T.);
#57355=EDGE_CURVE('',#43216,#40636,#35144,.T.);
#57356=EDGE_CURVE('',#41169,#43228,#35145,.T.);
#57357=EDGE_CURVE('',#43217,#40635,#35146,.T.);
#57358=EDGE_CURVE('',#43218,#41791,#35147,.T.);
#57359=EDGE_CURVE('',#43219,#41787,#2380,.T.);
#57360=EDGE_CURVE('',#40813,#43215,#35148,.T.);
#57361=EDGE_CURVE('',#43220,#41786,#35149,.T.);
#57362=EDGE_CURVE('',#40814,#43214,#35150,.T.);
#57363=EDGE_CURVE('',#43221,#41783,#35151,.T.);
#57364=EDGE_CURVE('',#41774,#43213,#35152,.T.);
#57365=EDGE_CURVE('',#43222,#41782,#35153,.T.);
#57366=EDGE_CURVE('',#41775,#43224,#2381,.T.);
#57367=EDGE_CURVE('',#43223,#41779,#35154,.T.);
#57368=EDGE_CURVE('',#43264,#41750,#2382,.T.);
#57369=EDGE_CURVE('',#41745,#43263,#35155,.T.);
#57370=EDGE_CURVE('',#41744,#43262,#35156,.T.);
#57371=EDGE_CURVE('',#43253,#41752,#35157,.T.);
#57372=EDGE_CURVE('',#41741,#43261,#35158,.T.);
#57373=EDGE_CURVE('',#43254,#40644,#35159,.T.);
#57374=EDGE_CURVE('',#41740,#43260,#35160,.T.);
#57375=EDGE_CURVE('',#43255,#40643,#35161,.T.);
#57376=EDGE_CURVE('',#41738,#43259,#2383,.T.);
#57377=EDGE_CURVE('',#43238,#40642,#35162,.T.);
#57378=EDGE_CURVE('',#41733,#43258,#35163,.T.);
#57379=EDGE_CURVE('',#43239,#40641,#35164,.T.);
#57380=EDGE_CURVE('',#41162,#43257,#35165,.T.);
#57381=EDGE_CURVE('',#43244,#40640,#35166,.T.);
#57382=EDGE_CURVE('',#41163,#43256,#35167,.T.);
#57383=EDGE_CURVE('',#43245,#40639,#35168,.T.);
#57384=EDGE_CURVE('',#41164,#43237,#35169,.T.);
#57385=EDGE_CURVE('',#43246,#41771,#35170,.T.);
#57386=EDGE_CURVE('',#41165,#43240,#35171,.T.);
#57387=EDGE_CURVE('',#43247,#41767,#2384,.T.);
#57388=EDGE_CURVE('',#41166,#43243,#35172,.T.);
#57389=EDGE_CURVE('',#43248,#41766,#35173,.T.);
#57390=EDGE_CURVE('',#41167,#43242,#35174,.T.);
#57391=EDGE_CURVE('',#43249,#41763,#35175,.T.);
#57392=EDGE_CURVE('',#41754,#43241,#35176,.T.);
#57393=EDGE_CURVE('',#43250,#41762,#35177,.T.);
#57394=EDGE_CURVE('',#41755,#43252,#2385,.T.);
#57395=EDGE_CURVE('',#43251,#41759,#35178,.T.);
#57396=EDGE_CURVE('',#43292,#41730,#2386,.T.);
#57397=EDGE_CURVE('',#41725,#43291,#35179,.T.);
#57398=EDGE_CURVE('',#41724,#43290,#35180,.T.);
#57399=EDGE_CURVE('',#43281,#41732,#35181,.T.);
#57400=EDGE_CURVE('',#41721,#43289,#35182,.T.);
#57401=EDGE_CURVE('',#43282,#40650,#35183,.T.);
#57402=EDGE_CURVE('',#41720,#43288,#35184,.T.);
#57403=EDGE_CURVE('',#43283,#40649,#35185,.T.);
#57404=EDGE_CURVE('',#41718,#43287,#2387,.T.);
#57405=EDGE_CURVE('',#43266,#40648,#35186,.T.);
#57406=EDGE_CURVE('',#41713,#43286,#35187,.T.);
#57407=EDGE_CURVE('',#43267,#40647,#35188,.T.);
#57408=EDGE_CURVE('',#41156,#43285,#35189,.T.);
#57409=EDGE_CURVE('',#43272,#40646,#35190,.T.);
#57410=EDGE_CURVE('',#41157,#43284,#35191,.T.);
#57411=EDGE_CURVE('',#43273,#40645,#35192,.T.);
#57412=EDGE_CURVE('',#41158,#43265,#35193,.T.);
#57413=EDGE_CURVE('',#43274,#41751,#35194,.T.);
#57414=EDGE_CURVE('',#41159,#43268,#35195,.T.);
#57415=EDGE_CURVE('',#43275,#41747,#2388,.T.);
#57416=EDGE_CURVE('',#41160,#43271,#35196,.T.);
#57417=EDGE_CURVE('',#43276,#41746,#35197,.T.);
#57418=EDGE_CURVE('',#41161,#43270,#35198,.T.);
#57419=EDGE_CURVE('',#43277,#41743,#35199,.T.);
#57420=EDGE_CURVE('',#41734,#43269,#35200,.T.);
#57421=EDGE_CURVE('',#43278,#41742,#35201,.T.);
#57422=EDGE_CURVE('',#41735,#43280,#2389,.T.);
#57423=EDGE_CURVE('',#43279,#41739,#35202,.T.);
#57424=EDGE_CURVE('',#43320,#41710,#2390,.T.);
#57425=EDGE_CURVE('',#41705,#43319,#35203,.T.);
#57426=EDGE_CURVE('',#41704,#43318,#35204,.T.);
#57427=EDGE_CURVE('',#43309,#41712,#35205,.T.);
#57428=EDGE_CURVE('',#41701,#43317,#35206,.T.);
#57429=EDGE_CURVE('',#43310,#40656,#35207,.T.);
#57430=EDGE_CURVE('',#41700,#43316,#35208,.T.);
#57431=EDGE_CURVE('',#43311,#40655,#35209,.T.);
#57432=EDGE_CURVE('',#41698,#43315,#2391,.T.);
#57433=EDGE_CURVE('',#43294,#40654,#35210,.T.);
#57434=EDGE_CURVE('',#41693,#43314,#35211,.T.);
#57435=EDGE_CURVE('',#43295,#40653,#35212,.T.);
#57436=EDGE_CURVE('',#41150,#43313,#35213,.T.);
#57437=EDGE_CURVE('',#43300,#40652,#35214,.T.);
#57438=EDGE_CURVE('',#41151,#43312,#35215,.T.);
#57439=EDGE_CURVE('',#43301,#40651,#35216,.T.);
#57440=EDGE_CURVE('',#41152,#43293,#35217,.T.);
#57441=EDGE_CURVE('',#43302,#41731,#35218,.T.);
#57442=EDGE_CURVE('',#41153,#43296,#35219,.T.);
#57443=EDGE_CURVE('',#43303,#41727,#2392,.T.);
#57444=EDGE_CURVE('',#41154,#43299,#35220,.T.);
#57445=EDGE_CURVE('',#43304,#41726,#35221,.T.);
#57446=EDGE_CURVE('',#41155,#43298,#35222,.T.);
#57447=EDGE_CURVE('',#43305,#41723,#35223,.T.);
#57448=EDGE_CURVE('',#41714,#43297,#35224,.T.);
#57449=EDGE_CURVE('',#43306,#41722,#35225,.T.);
#57450=EDGE_CURVE('',#41715,#43308,#2393,.T.);
#57451=EDGE_CURVE('',#43307,#41719,#35226,.T.);
#57452=EDGE_CURVE('',#43348,#41690,#2394,.T.);
#57453=EDGE_CURVE('',#41685,#43347,#35227,.T.);
#57454=EDGE_CURVE('',#41684,#43346,#35228,.T.);
#57455=EDGE_CURVE('',#43337,#41692,#35229,.T.);
#57456=EDGE_CURVE('',#41681,#43345,#35230,.T.);
#57457=EDGE_CURVE('',#43338,#40662,#35231,.T.);
#57458=EDGE_CURVE('',#41680,#43344,#35232,.T.);
#57459=EDGE_CURVE('',#43339,#40661,#35233,.T.);
#57460=EDGE_CURVE('',#41678,#43343,#2395,.T.);
#57461=EDGE_CURVE('',#43322,#40660,#35234,.T.);
#57462=EDGE_CURVE('',#41673,#43342,#35235,.T.);
#57463=EDGE_CURVE('',#43323,#40659,#35236,.T.);
#57464=EDGE_CURVE('',#41144,#43341,#35237,.T.);
#57465=EDGE_CURVE('',#43328,#40658,#35238,.T.);
#57466=EDGE_CURVE('',#41145,#43340,#35239,.T.);
#57467=EDGE_CURVE('',#43329,#40657,#35240,.T.);
#57468=EDGE_CURVE('',#41146,#43321,#35241,.T.);
#57469=EDGE_CURVE('',#43330,#41711,#35242,.T.);
#57470=EDGE_CURVE('',#41147,#43324,#35243,.T.);
#57471=EDGE_CURVE('',#43331,#41707,#2396,.T.);
#57472=EDGE_CURVE('',#41148,#43327,#35244,.T.);
#57473=EDGE_CURVE('',#43332,#41706,#35245,.T.);
#57474=EDGE_CURVE('',#41149,#43326,#35246,.T.);
#57475=EDGE_CURVE('',#43333,#41703,#35247,.T.);
#57476=EDGE_CURVE('',#41694,#43325,#35248,.T.);
#57477=EDGE_CURVE('',#43334,#41702,#35249,.T.);
#57478=EDGE_CURVE('',#41695,#43336,#2397,.T.);
#57479=EDGE_CURVE('',#43335,#41699,#35250,.T.);
#57480=EDGE_CURVE('',#43376,#41670,#2398,.T.);
#57481=EDGE_CURVE('',#41665,#43375,#35251,.T.);
#57482=EDGE_CURVE('',#41664,#43374,#35252,.T.);
#57483=EDGE_CURVE('',#43365,#41672,#35253,.T.);
#57484=EDGE_CURVE('',#41661,#43373,#35254,.T.);
#57485=EDGE_CURVE('',#43366,#40668,#35255,.T.);
#57486=EDGE_CURVE('',#41660,#43372,#35256,.T.);
#57487=EDGE_CURVE('',#43367,#40667,#35257,.T.);
#57488=EDGE_CURVE('',#41658,#43371,#2399,.T.);
#57489=EDGE_CURVE('',#43350,#40666,#35258,.T.);
#57490=EDGE_CURVE('',#41653,#43370,#35259,.T.);
#57491=EDGE_CURVE('',#43351,#40665,#35260,.T.);
#57492=EDGE_CURVE('',#41138,#43369,#35261,.T.);
#57493=EDGE_CURVE('',#43356,#40664,#35262,.T.);
#57494=EDGE_CURVE('',#41139,#43368,#35263,.T.);
#57495=EDGE_CURVE('',#43357,#40663,#35264,.T.);
#57496=EDGE_CURVE('',#41140,#43349,#35265,.T.);
#57497=EDGE_CURVE('',#43358,#41691,#35266,.T.);
#57498=EDGE_CURVE('',#41141,#43352,#35267,.T.);
#57499=EDGE_CURVE('',#43359,#41687,#2400,.T.);
#57500=EDGE_CURVE('',#41142,#43355,#35268,.T.);
#57501=EDGE_CURVE('',#43360,#41686,#35269,.T.);
#57502=EDGE_CURVE('',#41143,#43354,#35270,.T.);
#57503=EDGE_CURVE('',#43361,#41683,#35271,.T.);
#57504=EDGE_CURVE('',#41674,#43353,#35272,.T.);
#57505=EDGE_CURVE('',#43362,#41682,#35273,.T.);
#57506=EDGE_CURVE('',#41675,#43364,#2401,.T.);
#57507=EDGE_CURVE('',#43363,#41679,#35274,.T.);
#57508=EDGE_CURVE('',#43404,#41650,#2402,.T.);
#57509=EDGE_CURVE('',#41645,#43403,#35275,.T.);
#57510=EDGE_CURVE('',#41644,#43402,#35276,.T.);
#57511=EDGE_CURVE('',#43393,#41652,#35277,.T.);
#57512=EDGE_CURVE('',#41641,#43401,#35278,.T.);
#57513=EDGE_CURVE('',#43394,#40674,#35279,.T.);
#57514=EDGE_CURVE('',#41640,#43400,#35280,.T.);
#57515=EDGE_CURVE('',#43395,#40673,#35281,.T.);
#57516=EDGE_CURVE('',#41638,#43399,#2403,.T.);
#57517=EDGE_CURVE('',#43378,#40672,#35282,.T.);
#57518=EDGE_CURVE('',#41633,#43398,#35283,.T.);
#57519=EDGE_CURVE('',#43379,#40671,#35284,.T.);
#57520=EDGE_CURVE('',#41132,#43397,#35285,.T.);
#57521=EDGE_CURVE('',#43384,#40670,#35286,.T.);
#57522=EDGE_CURVE('',#41133,#43396,#35287,.T.);
#57523=EDGE_CURVE('',#43385,#40669,#35288,.T.);
#57524=EDGE_CURVE('',#41134,#43377,#35289,.T.);
#57525=EDGE_CURVE('',#43386,#41671,#35290,.T.);
#57526=EDGE_CURVE('',#41135,#43380,#35291,.T.);
#57527=EDGE_CURVE('',#43387,#41667,#2404,.T.);
#57528=EDGE_CURVE('',#41136,#43383,#35292,.T.);
#57529=EDGE_CURVE('',#43388,#41666,#35293,.T.);
#57530=EDGE_CURVE('',#41137,#43382,#35294,.T.);
#57531=EDGE_CURVE('',#43389,#41663,#35295,.T.);
#57532=EDGE_CURVE('',#41654,#43381,#35296,.T.);
#57533=EDGE_CURVE('',#43390,#41662,#35297,.T.);
#57534=EDGE_CURVE('',#41655,#43392,#2405,.T.);
#57535=EDGE_CURVE('',#43391,#41659,#35298,.T.);
#57536=EDGE_CURVE('',#43432,#41630,#2406,.T.);
#57537=EDGE_CURVE('',#41625,#43431,#35299,.T.);
#57538=EDGE_CURVE('',#41624,#43430,#35300,.T.);
#57539=EDGE_CURVE('',#43421,#41632,#35301,.T.);
#57540=EDGE_CURVE('',#41621,#43429,#35302,.T.);
#57541=EDGE_CURVE('',#43422,#40680,#35303,.T.);
#57542=EDGE_CURVE('',#41620,#43428,#35304,.T.);
#57543=EDGE_CURVE('',#43423,#40679,#35305,.T.);
#57544=EDGE_CURVE('',#41618,#43427,#2407,.T.);
#57545=EDGE_CURVE('',#43406,#40678,#35306,.T.);
#57546=EDGE_CURVE('',#41613,#43426,#35307,.T.);
#57547=EDGE_CURVE('',#43407,#40677,#35308,.T.);
#57548=EDGE_CURVE('',#41126,#43425,#35309,.T.);
#57549=EDGE_CURVE('',#43412,#40676,#35310,.T.);
#57550=EDGE_CURVE('',#41127,#43424,#35311,.T.);
#57551=EDGE_CURVE('',#43413,#40675,#35312,.T.);
#57552=EDGE_CURVE('',#41128,#43405,#35313,.T.);
#57553=EDGE_CURVE('',#43414,#41651,#35314,.T.);
#57554=EDGE_CURVE('',#41129,#43408,#35315,.T.);
#57555=EDGE_CURVE('',#43415,#41647,#2408,.T.);
#57556=EDGE_CURVE('',#41130,#43411,#35316,.T.);
#57557=EDGE_CURVE('',#43416,#41646,#35317,.T.);
#57558=EDGE_CURVE('',#41131,#43410,#35318,.T.);
#57559=EDGE_CURVE('',#43417,#41643,#35319,.T.);
#57560=EDGE_CURVE('',#41634,#43409,#35320,.T.);
#57561=EDGE_CURVE('',#43418,#41642,#35321,.T.);
#57562=EDGE_CURVE('',#41635,#43420,#2409,.T.);
#57563=EDGE_CURVE('',#43419,#41639,#35322,.T.);
#57564=EDGE_CURVE('',#43460,#41610,#2410,.T.);
#57565=EDGE_CURVE('',#41605,#43459,#35323,.T.);
#57566=EDGE_CURVE('',#41604,#43458,#35324,.T.);
#57567=EDGE_CURVE('',#43449,#41612,#35325,.T.);
#57568=EDGE_CURVE('',#41601,#43457,#35326,.T.);
#57569=EDGE_CURVE('',#43450,#40686,#35327,.T.);
#57570=EDGE_CURVE('',#41600,#43456,#35328,.T.);
#57571=EDGE_CURVE('',#43451,#40685,#35329,.T.);
#57572=EDGE_CURVE('',#41598,#43455,#2411,.T.);
#57573=EDGE_CURVE('',#43434,#40684,#35330,.T.);
#57574=EDGE_CURVE('',#41593,#43454,#35331,.T.);
#57575=EDGE_CURVE('',#43435,#40683,#35332,.T.);
#57576=EDGE_CURVE('',#41120,#43453,#35333,.T.);
#57577=EDGE_CURVE('',#43440,#40682,#35334,.T.);
#57578=EDGE_CURVE('',#41121,#43452,#35335,.T.);
#57579=EDGE_CURVE('',#43441,#40681,#35336,.T.);
#57580=EDGE_CURVE('',#41122,#43433,#35337,.T.);
#57581=EDGE_CURVE('',#43442,#41631,#35338,.T.);
#57582=EDGE_CURVE('',#41123,#43436,#35339,.T.);
#57583=EDGE_CURVE('',#43443,#41627,#2412,.T.);
#57584=EDGE_CURVE('',#41124,#43439,#35340,.T.);
#57585=EDGE_CURVE('',#43444,#41626,#35341,.T.);
#57586=EDGE_CURVE('',#41125,#43438,#35342,.T.);
#57587=EDGE_CURVE('',#43445,#41623,#35343,.T.);
#57588=EDGE_CURVE('',#41614,#43437,#35344,.T.);
#57589=EDGE_CURVE('',#43446,#41622,#35345,.T.);
#57590=EDGE_CURVE('',#41615,#43448,#2413,.T.);
#57591=EDGE_CURVE('',#43447,#41619,#35346,.T.);
#57592=EDGE_CURVE('',#43488,#41590,#2414,.T.);
#57593=EDGE_CURVE('',#41585,#43487,#35347,.T.);
#57594=EDGE_CURVE('',#41584,#43486,#35348,.T.);
#57595=EDGE_CURVE('',#43477,#41592,#35349,.T.);
#57596=EDGE_CURVE('',#41581,#43485,#35350,.T.);
#57597=EDGE_CURVE('',#43478,#40692,#35351,.T.);
#57598=EDGE_CURVE('',#41580,#43484,#35352,.T.);
#57599=EDGE_CURVE('',#43479,#40691,#35353,.T.);
#57600=EDGE_CURVE('',#41578,#43483,#2415,.T.);
#57601=EDGE_CURVE('',#43462,#40690,#35354,.T.);
#57602=EDGE_CURVE('',#41573,#43482,#35355,.T.);
#57603=EDGE_CURVE('',#43463,#40689,#35356,.T.);
#57604=EDGE_CURVE('',#41114,#43481,#35357,.T.);
#57605=EDGE_CURVE('',#43468,#40688,#35358,.T.);
#57606=EDGE_CURVE('',#41115,#43480,#35359,.T.);
#57607=EDGE_CURVE('',#43469,#40687,#35360,.T.);
#57608=EDGE_CURVE('',#41116,#43461,#35361,.T.);
#57609=EDGE_CURVE('',#43470,#41611,#35362,.T.);
#57610=EDGE_CURVE('',#41117,#43464,#35363,.T.);
#57611=EDGE_CURVE('',#43471,#41607,#2416,.T.);
#57612=EDGE_CURVE('',#41118,#43467,#35364,.T.);
#57613=EDGE_CURVE('',#43472,#41606,#35365,.T.);
#57614=EDGE_CURVE('',#41119,#43466,#35366,.T.);
#57615=EDGE_CURVE('',#43473,#41603,#35367,.T.);
#57616=EDGE_CURVE('',#41594,#43465,#35368,.T.);
#57617=EDGE_CURVE('',#43474,#41602,#35369,.T.);
#57618=EDGE_CURVE('',#41595,#43476,#2417,.T.);
#57619=EDGE_CURVE('',#43475,#41599,#35370,.T.);
#57620=EDGE_CURVE('',#43516,#41570,#2418,.T.);
#57621=EDGE_CURVE('',#41565,#43515,#35371,.T.);
#57622=EDGE_CURVE('',#41564,#43514,#35372,.T.);
#57623=EDGE_CURVE('',#43505,#41572,#35373,.T.);
#57624=EDGE_CURVE('',#41561,#43513,#35374,.T.);
#57625=EDGE_CURVE('',#43506,#40698,#35375,.T.);
#57626=EDGE_CURVE('',#41560,#43512,#35376,.T.);
#57627=EDGE_CURVE('',#43507,#40697,#35377,.T.);
#57628=EDGE_CURVE('',#41558,#43511,#2419,.T.);
#57629=EDGE_CURVE('',#43490,#40696,#35378,.T.);
#57630=EDGE_CURVE('',#41553,#43510,#35379,.T.);
#57631=EDGE_CURVE('',#43491,#40695,#35380,.T.);
#57632=EDGE_CURVE('',#41108,#43509,#35381,.T.);
#57633=EDGE_CURVE('',#43496,#40694,#35382,.T.);
#57634=EDGE_CURVE('',#41109,#43508,#35383,.T.);
#57635=EDGE_CURVE('',#43497,#40693,#35384,.T.);
#57636=EDGE_CURVE('',#41110,#43489,#35385,.T.);
#57637=EDGE_CURVE('',#43498,#41591,#35386,.T.);
#57638=EDGE_CURVE('',#41111,#43492,#35387,.T.);
#57639=EDGE_CURVE('',#43499,#41587,#2420,.T.);
#57640=EDGE_CURVE('',#41112,#43495,#35388,.T.);
#57641=EDGE_CURVE('',#43500,#41586,#35389,.T.);
#57642=EDGE_CURVE('',#41113,#43494,#35390,.T.);
#57643=EDGE_CURVE('',#43501,#41583,#35391,.T.);
#57644=EDGE_CURVE('',#41574,#43493,#35392,.T.);
#57645=EDGE_CURVE('',#43502,#41582,#35393,.T.);
#57646=EDGE_CURVE('',#41575,#43504,#2421,.T.);
#57647=EDGE_CURVE('',#43503,#41579,#35394,.T.);
#57648=EDGE_CURVE('',#43544,#41550,#2422,.T.);
#57649=EDGE_CURVE('',#41545,#43543,#35395,.T.);
#57650=EDGE_CURVE('',#41544,#43542,#35396,.T.);
#57651=EDGE_CURVE('',#43533,#41552,#35397,.T.);
#57652=EDGE_CURVE('',#41541,#43541,#35398,.T.);
#57653=EDGE_CURVE('',#43534,#40704,#35399,.T.);
#57654=EDGE_CURVE('',#41540,#43540,#35400,.T.);
#57655=EDGE_CURVE('',#43535,#40703,#35401,.T.);
#57656=EDGE_CURVE('',#41538,#43539,#2423,.T.);
#57657=EDGE_CURVE('',#43518,#40702,#35402,.T.);
#57658=EDGE_CURVE('',#41533,#43538,#35403,.T.);
#57659=EDGE_CURVE('',#43519,#40701,#35404,.T.);
#57660=EDGE_CURVE('',#41102,#43537,#35405,.T.);
#57661=EDGE_CURVE('',#43524,#40700,#35406,.T.);
#57662=EDGE_CURVE('',#41103,#43536,#35407,.T.);
#57663=EDGE_CURVE('',#43525,#40699,#35408,.T.);
#57664=EDGE_CURVE('',#41104,#43517,#35409,.T.);
#57665=EDGE_CURVE('',#43526,#41571,#35410,.T.);
#57666=EDGE_CURVE('',#41105,#43520,#35411,.T.);
#57667=EDGE_CURVE('',#43527,#41567,#2424,.T.);
#57668=EDGE_CURVE('',#41106,#43523,#35412,.T.);
#57669=EDGE_CURVE('',#43528,#41566,#35413,.T.);
#57670=EDGE_CURVE('',#41107,#43522,#35414,.T.);
#57671=EDGE_CURVE('',#43529,#41563,#35415,.T.);
#57672=EDGE_CURVE('',#41554,#43521,#35416,.T.);
#57673=EDGE_CURVE('',#43530,#41562,#35417,.T.);
#57674=EDGE_CURVE('',#41555,#43532,#2425,.T.);
#57675=EDGE_CURVE('',#43531,#41559,#35418,.T.);
#57676=EDGE_CURVE('',#43572,#41530,#2426,.T.);
#57677=EDGE_CURVE('',#41525,#43571,#35419,.T.);
#57678=EDGE_CURVE('',#41524,#43570,#35420,.T.);
#57679=EDGE_CURVE('',#43561,#41532,#35421,.T.);
#57680=EDGE_CURVE('',#41521,#43569,#35422,.T.);
#57681=EDGE_CURVE('',#43562,#40710,#35423,.T.);
#57682=EDGE_CURVE('',#41520,#43568,#35424,.T.);
#57683=EDGE_CURVE('',#43563,#40709,#35425,.T.);
#57684=EDGE_CURVE('',#41518,#43567,#2427,.T.);
#57685=EDGE_CURVE('',#43546,#40708,#35426,.T.);
#57686=EDGE_CURVE('',#41513,#43566,#35427,.T.);
#57687=EDGE_CURVE('',#43547,#40707,#35428,.T.);
#57688=EDGE_CURVE('',#41096,#43565,#35429,.T.);
#57689=EDGE_CURVE('',#43552,#40706,#35430,.T.);
#57690=EDGE_CURVE('',#41097,#43564,#35431,.T.);
#57691=EDGE_CURVE('',#43553,#40705,#35432,.T.);
#57692=EDGE_CURVE('',#41098,#43545,#35433,.T.);
#57693=EDGE_CURVE('',#43554,#41551,#35434,.T.);
#57694=EDGE_CURVE('',#41099,#43548,#35435,.T.);
#57695=EDGE_CURVE('',#43555,#41547,#2428,.T.);
#57696=EDGE_CURVE('',#41100,#43551,#35436,.T.);
#57697=EDGE_CURVE('',#43556,#41546,#35437,.T.);
#57698=EDGE_CURVE('',#41101,#43550,#35438,.T.);
#57699=EDGE_CURVE('',#43557,#41543,#35439,.T.);
#57700=EDGE_CURVE('',#41534,#43549,#35440,.T.);
#57701=EDGE_CURVE('',#43558,#41542,#35441,.T.);
#57702=EDGE_CURVE('',#41535,#43560,#2429,.T.);
#57703=EDGE_CURVE('',#43559,#41539,#35442,.T.);
#57704=EDGE_CURVE('',#43600,#41510,#2430,.T.);
#57705=EDGE_CURVE('',#41505,#43599,#35443,.T.);
#57706=EDGE_CURVE('',#41504,#43598,#35444,.T.);
#57707=EDGE_CURVE('',#43589,#41512,#35445,.T.);
#57708=EDGE_CURVE('',#41501,#43597,#35446,.T.);
#57709=EDGE_CURVE('',#43590,#40716,#35447,.T.);
#57710=EDGE_CURVE('',#41500,#43596,#35448,.T.);
#57711=EDGE_CURVE('',#43591,#40715,#35449,.T.);
#57712=EDGE_CURVE('',#41498,#43595,#2431,.T.);
#57713=EDGE_CURVE('',#43574,#40714,#35450,.T.);
#57714=EDGE_CURVE('',#41493,#43594,#35451,.T.);
#57715=EDGE_CURVE('',#43575,#40713,#35452,.T.);
#57716=EDGE_CURVE('',#41090,#43593,#35453,.T.);
#57717=EDGE_CURVE('',#43580,#40712,#35454,.T.);
#57718=EDGE_CURVE('',#41091,#43592,#35455,.T.);
#57719=EDGE_CURVE('',#43581,#40711,#35456,.T.);
#57720=EDGE_CURVE('',#41092,#43573,#35457,.T.);
#57721=EDGE_CURVE('',#43582,#41531,#35458,.T.);
#57722=EDGE_CURVE('',#41093,#43576,#35459,.T.);
#57723=EDGE_CURVE('',#43583,#41527,#2432,.T.);
#57724=EDGE_CURVE('',#41094,#43579,#35460,.T.);
#57725=EDGE_CURVE('',#43584,#41526,#35461,.T.);
#57726=EDGE_CURVE('',#41095,#43578,#35462,.T.);
#57727=EDGE_CURVE('',#43585,#41523,#35463,.T.);
#57728=EDGE_CURVE('',#41514,#43577,#35464,.T.);
#57729=EDGE_CURVE('',#43586,#41522,#35465,.T.);
#57730=EDGE_CURVE('',#41515,#43588,#2433,.T.);
#57731=EDGE_CURVE('',#43587,#41519,#35466,.T.);
#57732=EDGE_CURVE('',#43628,#41490,#2434,.T.);
#57733=EDGE_CURVE('',#41485,#43627,#35467,.T.);
#57734=EDGE_CURVE('',#41484,#43626,#35468,.T.);
#57735=EDGE_CURVE('',#43617,#41492,#35469,.T.);
#57736=EDGE_CURVE('',#41481,#43625,#35470,.T.);
#57737=EDGE_CURVE('',#43618,#40722,#35471,.T.);
#57738=EDGE_CURVE('',#41480,#43624,#35472,.T.);
#57739=EDGE_CURVE('',#43619,#40721,#35473,.T.);
#57740=EDGE_CURVE('',#41478,#43623,#2435,.T.);
#57741=EDGE_CURVE('',#43602,#40720,#35474,.T.);
#57742=EDGE_CURVE('',#41473,#43622,#35475,.T.);
#57743=EDGE_CURVE('',#43603,#40719,#35476,.T.);
#57744=EDGE_CURVE('',#41084,#43621,#35477,.T.);
#57745=EDGE_CURVE('',#43608,#40718,#35478,.T.);
#57746=EDGE_CURVE('',#41085,#43620,#35479,.T.);
#57747=EDGE_CURVE('',#43609,#40717,#35480,.T.);
#57748=EDGE_CURVE('',#41086,#43601,#35481,.T.);
#57749=EDGE_CURVE('',#43610,#41511,#35482,.T.);
#57750=EDGE_CURVE('',#41087,#43604,#35483,.T.);
#57751=EDGE_CURVE('',#43611,#41507,#2436,.T.);
#57752=EDGE_CURVE('',#41088,#43607,#35484,.T.);
#57753=EDGE_CURVE('',#43612,#41506,#35485,.T.);
#57754=EDGE_CURVE('',#41089,#43606,#35486,.T.);
#57755=EDGE_CURVE('',#43613,#41503,#35487,.T.);
#57756=EDGE_CURVE('',#41494,#43605,#35488,.T.);
#57757=EDGE_CURVE('',#43614,#41502,#35489,.T.);
#57758=EDGE_CURVE('',#41495,#43616,#2437,.T.);
#57759=EDGE_CURVE('',#43615,#41499,#35490,.T.);
#57760=EDGE_CURVE('',#43652,#41470,#2438,.T.);
#57761=EDGE_CURVE('',#41465,#43651,#35491,.T.);
#57762=EDGE_CURVE('',#41464,#43650,#35492,.T.);
#57763=EDGE_CURVE('',#43641,#41472,#35493,.T.);
#57764=EDGE_CURVE('',#41461,#43649,#35494,.T.);
#57765=EDGE_CURVE('',#43642,#40726,#35495,.T.);
#57766=EDGE_CURVE('',#41460,#43648,#35496,.T.);
#57767=EDGE_CURVE('',#43643,#40725,#35497,.T.);
#57768=EDGE_CURVE('',#41458,#43647,#2439,.T.);
#57769=EDGE_CURVE('',#41453,#43646,#35498,.T.);
#57770=EDGE_CURVE('',#41080,#43645,#35499,.T.);
#57771=EDGE_CURVE('',#43632,#40724,#35500,.T.);
#57772=EDGE_CURVE('',#41081,#43644,#35501,.T.);
#57773=EDGE_CURVE('',#43633,#40723,#35502,.T.);
#57774=EDGE_CURVE('',#43634,#41491,#35503,.T.);
#57775=EDGE_CURVE('',#43635,#41487,#2440,.T.);
#57776=EDGE_CURVE('',#41082,#43631,#35504,.T.);
#57777=EDGE_CURVE('',#43636,#41486,#35505,.T.);
#57778=EDGE_CURVE('',#41083,#43630,#35506,.T.);
#57779=EDGE_CURVE('',#43637,#41483,#35507,.T.);
#57780=EDGE_CURVE('',#41474,#43629,#35508,.T.);
#57781=EDGE_CURVE('',#43638,#41482,#35509,.T.);
#57782=EDGE_CURVE('',#41475,#43640,#2441,.T.);
#57783=EDGE_CURVE('',#43639,#41479,#35510,.T.);
#57784=EDGE_CURVE('',#43680,#41450,#2442,.T.);
#57785=EDGE_CURVE('',#41445,#43679,#35511,.T.);
#57786=EDGE_CURVE('',#41444,#43678,#35512,.T.);
#57787=EDGE_CURVE('',#43669,#41452,#35513,.T.);
#57788=EDGE_CURVE('',#41441,#43677,#35514,.T.);
#57789=EDGE_CURVE('',#43670,#40732,#35515,.T.);
#57790=EDGE_CURVE('',#41440,#43676,#35516,.T.);
#57791=EDGE_CURVE('',#43671,#40731,#35517,.T.);
#57792=EDGE_CURVE('',#41438,#43675,#2443,.T.);
#57793=EDGE_CURVE('',#43654,#40730,#35518,.T.);
#57794=EDGE_CURVE('',#41433,#43674,#35519,.T.);
#57795=EDGE_CURVE('',#43655,#40729,#35520,.T.);
#57796=EDGE_CURVE('',#41074,#43673,#35521,.T.);
#57797=EDGE_CURVE('',#43660,#40728,#35522,.T.);
#57798=EDGE_CURVE('',#41075,#43672,#35523,.T.);
#57799=EDGE_CURVE('',#43661,#40727,#35524,.T.);
#57800=EDGE_CURVE('',#41076,#43653,#35525,.T.);
#57801=EDGE_CURVE('',#43662,#41471,#35526,.T.);
#57802=EDGE_CURVE('',#41077,#43656,#35527,.T.);
#57803=EDGE_CURVE('',#43663,#41467,#2444,.T.);
#57804=EDGE_CURVE('',#41078,#43659,#35528,.T.);
#57805=EDGE_CURVE('',#43664,#41466,#35529,.T.);
#57806=EDGE_CURVE('',#41079,#43658,#35530,.T.);
#57807=EDGE_CURVE('',#43665,#41463,#35531,.T.);
#57808=EDGE_CURVE('',#41454,#43657,#35532,.T.);
#57809=EDGE_CURVE('',#43666,#41462,#35533,.T.);
#57810=EDGE_CURVE('',#41455,#43668,#2445,.T.);
#57811=EDGE_CURVE('',#43667,#41459,#35534,.T.);
#57812=EDGE_CURVE('',#43708,#41430,#2446,.T.);
#57813=EDGE_CURVE('',#41425,#43707,#35535,.T.);
#57814=EDGE_CURVE('',#41424,#43706,#35536,.T.);
#57815=EDGE_CURVE('',#43697,#41432,#35537,.T.);
#57816=EDGE_CURVE('',#41421,#43705,#35538,.T.);
#57817=EDGE_CURVE('',#43698,#40738,#35539,.T.);
#57818=EDGE_CURVE('',#41420,#43704,#35540,.T.);
#57819=EDGE_CURVE('',#43699,#40737,#35541,.T.);
#57820=EDGE_CURVE('',#41418,#43703,#2447,.T.);
#57821=EDGE_CURVE('',#43682,#40736,#35542,.T.);
#57822=EDGE_CURVE('',#41413,#43702,#35543,.T.);
#57823=EDGE_CURVE('',#43683,#40735,#35544,.T.);
#57824=EDGE_CURVE('',#41068,#43701,#35545,.T.);
#57825=EDGE_CURVE('',#43688,#40734,#35546,.T.);
#57826=EDGE_CURVE('',#41069,#43700,#35547,.T.);
#57827=EDGE_CURVE('',#43689,#40733,#35548,.T.);
#57828=EDGE_CURVE('',#41070,#43681,#35549,.T.);
#57829=EDGE_CURVE('',#43690,#41451,#35550,.T.);
#57830=EDGE_CURVE('',#41071,#43684,#35551,.T.);
#57831=EDGE_CURVE('',#43691,#41447,#2448,.T.);
#57832=EDGE_CURVE('',#41072,#43687,#35552,.T.);
#57833=EDGE_CURVE('',#43692,#41446,#35553,.T.);
#57834=EDGE_CURVE('',#41073,#43686,#35554,.T.);
#57835=EDGE_CURVE('',#43693,#41443,#35555,.T.);
#57836=EDGE_CURVE('',#41434,#43685,#35556,.T.);
#57837=EDGE_CURVE('',#43694,#41442,#35557,.T.);
#57838=EDGE_CURVE('',#41435,#43696,#2449,.T.);
#57839=EDGE_CURVE('',#43695,#41439,#35558,.T.);
#57840=EDGE_CURVE('',#43736,#41410,#2450,.T.);
#57841=EDGE_CURVE('',#41405,#43735,#35559,.T.);
#57842=EDGE_CURVE('',#41404,#43734,#35560,.T.);
#57843=EDGE_CURVE('',#43725,#41412,#35561,.T.);
#57844=EDGE_CURVE('',#41401,#43733,#35562,.T.);
#57845=EDGE_CURVE('',#43726,#40744,#35563,.T.);
#57846=EDGE_CURVE('',#41400,#43732,#35564,.T.);
#57847=EDGE_CURVE('',#43727,#40743,#35565,.T.);
#57848=EDGE_CURVE('',#41398,#43731,#2451,.T.);
#57849=EDGE_CURVE('',#43710,#40742,#35566,.T.);
#57850=EDGE_CURVE('',#41393,#43730,#35567,.T.);
#57851=EDGE_CURVE('',#43711,#40741,#35568,.T.);
#57852=EDGE_CURVE('',#41062,#43729,#35569,.T.);
#57853=EDGE_CURVE('',#43716,#40740,#35570,.T.);
#57854=EDGE_CURVE('',#41063,#43728,#35571,.T.);
#57855=EDGE_CURVE('',#43717,#40739,#35572,.T.);
#57856=EDGE_CURVE('',#41064,#43709,#35573,.T.);
#57857=EDGE_CURVE('',#43718,#41431,#35574,.T.);
#57858=EDGE_CURVE('',#41065,#43712,#35575,.T.);
#57859=EDGE_CURVE('',#43719,#41427,#2452,.T.);
#57860=EDGE_CURVE('',#41066,#43715,#35576,.T.);
#57861=EDGE_CURVE('',#43720,#41426,#35577,.T.);
#57862=EDGE_CURVE('',#41067,#43714,#35578,.T.);
#57863=EDGE_CURVE('',#43721,#41423,#35579,.T.);
#57864=EDGE_CURVE('',#41414,#43713,#35580,.T.);
#57865=EDGE_CURVE('',#43722,#41422,#35581,.T.);
#57866=EDGE_CURVE('',#41415,#43724,#2453,.T.);
#57867=EDGE_CURVE('',#43723,#41419,#35582,.T.);
#57868=EDGE_CURVE('',#43764,#41390,#2454,.T.);
#57869=EDGE_CURVE('',#41385,#43763,#35583,.T.);
#57870=EDGE_CURVE('',#41384,#43762,#35584,.T.);
#57871=EDGE_CURVE('',#43753,#41392,#35585,.T.);
#57872=EDGE_CURVE('',#41381,#43761,#35586,.T.);
#57873=EDGE_CURVE('',#43754,#40750,#35587,.T.);
#57874=EDGE_CURVE('',#41380,#43760,#35588,.T.);
#57875=EDGE_CURVE('',#43755,#40749,#35589,.T.);
#57876=EDGE_CURVE('',#41378,#43759,#2455,.T.);
#57877=EDGE_CURVE('',#43738,#40748,#35590,.T.);
#57878=EDGE_CURVE('',#41373,#43758,#35591,.T.);
#57879=EDGE_CURVE('',#43739,#40747,#35592,.T.);
#57880=EDGE_CURVE('',#41056,#43757,#35593,.T.);
#57881=EDGE_CURVE('',#43744,#40746,#35594,.T.);
#57882=EDGE_CURVE('',#41057,#43756,#35595,.T.);
#57883=EDGE_CURVE('',#43745,#40745,#35596,.T.);
#57884=EDGE_CURVE('',#41058,#43737,#35597,.T.);
#57885=EDGE_CURVE('',#43746,#41411,#35598,.T.);
#57886=EDGE_CURVE('',#41059,#43740,#35599,.T.);
#57887=EDGE_CURVE('',#43747,#41407,#2456,.T.);
#57888=EDGE_CURVE('',#41060,#43743,#35600,.T.);
#57889=EDGE_CURVE('',#43748,#41406,#35601,.T.);
#57890=EDGE_CURVE('',#41061,#43742,#35602,.T.);
#57891=EDGE_CURVE('',#43749,#41403,#35603,.T.);
#57892=EDGE_CURVE('',#41394,#43741,#35604,.T.);
#57893=EDGE_CURVE('',#43750,#41402,#35605,.T.);
#57894=EDGE_CURVE('',#41395,#43752,#2457,.T.);
#57895=EDGE_CURVE('',#43751,#41399,#35606,.T.);
#57896=EDGE_CURVE('',#43792,#41370,#2458,.T.);
#57897=EDGE_CURVE('',#41365,#43791,#35607,.T.);
#57898=EDGE_CURVE('',#41364,#43790,#35608,.T.);
#57899=EDGE_CURVE('',#43781,#41372,#35609,.T.);
#57900=EDGE_CURVE('',#41361,#43789,#35610,.T.);
#57901=EDGE_CURVE('',#43782,#40756,#35611,.T.);
#57902=EDGE_CURVE('',#41360,#43788,#35612,.T.);
#57903=EDGE_CURVE('',#43783,#40755,#35613,.T.);
#57904=EDGE_CURVE('',#41358,#43787,#2459,.T.);
#57905=EDGE_CURVE('',#43766,#40754,#35614,.T.);
#57906=EDGE_CURVE('',#41353,#43786,#35615,.T.);
#57907=EDGE_CURVE('',#43767,#40753,#35616,.T.);
#57908=EDGE_CURVE('',#41050,#43785,#35617,.T.);
#57909=EDGE_CURVE('',#43772,#40752,#35618,.T.);
#57910=EDGE_CURVE('',#41051,#43784,#35619,.T.);
#57911=EDGE_CURVE('',#43773,#40751,#35620,.T.);
#57912=EDGE_CURVE('',#41052,#43765,#35621,.T.);
#57913=EDGE_CURVE('',#43774,#41391,#35622,.T.);
#57914=EDGE_CURVE('',#41053,#43768,#35623,.T.);
#57915=EDGE_CURVE('',#43775,#41387,#2460,.T.);
#57916=EDGE_CURVE('',#41054,#43771,#35624,.T.);
#57917=EDGE_CURVE('',#43776,#41386,#35625,.T.);
#57918=EDGE_CURVE('',#41055,#43770,#35626,.T.);
#57919=EDGE_CURVE('',#43777,#41383,#35627,.T.);
#57920=EDGE_CURVE('',#41374,#43769,#35628,.T.);
#57921=EDGE_CURVE('',#43778,#41382,#35629,.T.);
#57922=EDGE_CURVE('',#41375,#43780,#2461,.T.);
#57923=EDGE_CURVE('',#43779,#41379,#35630,.T.);
#57924=EDGE_CURVE('',#43820,#41350,#2462,.T.);
#57925=EDGE_CURVE('',#41345,#43819,#35631,.T.);
#57926=EDGE_CURVE('',#41344,#43818,#35632,.T.);
#57927=EDGE_CURVE('',#43809,#41352,#35633,.T.);
#57928=EDGE_CURVE('',#41341,#43817,#35634,.T.);
#57929=EDGE_CURVE('',#43810,#40762,#35635,.T.);
#57930=EDGE_CURVE('',#41340,#43816,#35636,.T.);
#57931=EDGE_CURVE('',#43811,#40761,#35637,.T.);
#57932=EDGE_CURVE('',#41338,#43815,#2463,.T.);
#57933=EDGE_CURVE('',#43794,#40760,#35638,.T.);
#57934=EDGE_CURVE('',#41333,#43814,#35639,.T.);
#57935=EDGE_CURVE('',#43795,#40759,#35640,.T.);
#57936=EDGE_CURVE('',#41044,#43813,#35641,.T.);
#57937=EDGE_CURVE('',#43800,#40758,#35642,.T.);
#57938=EDGE_CURVE('',#41045,#43812,#35643,.T.);
#57939=EDGE_CURVE('',#43801,#40757,#35644,.T.);
#57940=EDGE_CURVE('',#41046,#43793,#35645,.T.);
#57941=EDGE_CURVE('',#43802,#41371,#35646,.T.);
#57942=EDGE_CURVE('',#41047,#43796,#35647,.T.);
#57943=EDGE_CURVE('',#43803,#41367,#2464,.T.);
#57944=EDGE_CURVE('',#41048,#43799,#35648,.T.);
#57945=EDGE_CURVE('',#43804,#41366,#35649,.T.);
#57946=EDGE_CURVE('',#41049,#43798,#35650,.T.);
#57947=EDGE_CURVE('',#43805,#41363,#35651,.T.);
#57948=EDGE_CURVE('',#41354,#43797,#35652,.T.);
#57949=EDGE_CURVE('',#43806,#41362,#35653,.T.);
#57950=EDGE_CURVE('',#41355,#43808,#2465,.T.);
#57951=EDGE_CURVE('',#43807,#41359,#35654,.T.);
#57952=EDGE_CURVE('',#43848,#41330,#2466,.T.);
#57953=EDGE_CURVE('',#41325,#43847,#35655,.T.);
#57954=EDGE_CURVE('',#41324,#43846,#35656,.T.);
#57955=EDGE_CURVE('',#43837,#41332,#35657,.T.);
#57956=EDGE_CURVE('',#41321,#43845,#35658,.T.);
#57957=EDGE_CURVE('',#43838,#40768,#35659,.T.);
#57958=EDGE_CURVE('',#41320,#43844,#35660,.T.);
#57959=EDGE_CURVE('',#43839,#40767,#35661,.T.);
#57960=EDGE_CURVE('',#41318,#43843,#2467,.T.);
#57961=EDGE_CURVE('',#43822,#40766,#35662,.T.);
#57962=EDGE_CURVE('',#41313,#43842,#35663,.T.);
#57963=EDGE_CURVE('',#43823,#40765,#35664,.T.);
#57964=EDGE_CURVE('',#41038,#43841,#35665,.T.);
#57965=EDGE_CURVE('',#43828,#40764,#35666,.T.);
#57966=EDGE_CURVE('',#41039,#43840,#35667,.T.);
#57967=EDGE_CURVE('',#43829,#40763,#35668,.T.);
#57968=EDGE_CURVE('',#41040,#43821,#35669,.T.);
#57969=EDGE_CURVE('',#43830,#41351,#35670,.T.);
#57970=EDGE_CURVE('',#41041,#43824,#35671,.T.);
#57971=EDGE_CURVE('',#43831,#41347,#2468,.T.);
#57972=EDGE_CURVE('',#41042,#43827,#35672,.T.);
#57973=EDGE_CURVE('',#43832,#41346,#35673,.T.);
#57974=EDGE_CURVE('',#41043,#43826,#35674,.T.);
#57975=EDGE_CURVE('',#43833,#41343,#35675,.T.);
#57976=EDGE_CURVE('',#41334,#43825,#35676,.T.);
#57977=EDGE_CURVE('',#43834,#41342,#35677,.T.);
#57978=EDGE_CURVE('',#41335,#43836,#2469,.T.);
#57979=EDGE_CURVE('',#43835,#41339,#35678,.T.);
#57980=EDGE_CURVE('',#43876,#41310,#2470,.T.);
#57981=EDGE_CURVE('',#41305,#43875,#35679,.T.);
#57982=EDGE_CURVE('',#41304,#43874,#35680,.T.);
#57983=EDGE_CURVE('',#43865,#41312,#35681,.T.);
#57984=EDGE_CURVE('',#41301,#43873,#35682,.T.);
#57985=EDGE_CURVE('',#43866,#40774,#35683,.T.);
#57986=EDGE_CURVE('',#41300,#43872,#35684,.T.);
#57987=EDGE_CURVE('',#43867,#40773,#35685,.T.);
#57988=EDGE_CURVE('',#41298,#43871,#2471,.T.);
#57989=EDGE_CURVE('',#43850,#40772,#35686,.T.);
#57990=EDGE_CURVE('',#41293,#43870,#35687,.T.);
#57991=EDGE_CURVE('',#43851,#40771,#35688,.T.);
#57992=EDGE_CURVE('',#41032,#43869,#35689,.T.);
#57993=EDGE_CURVE('',#43856,#40770,#35690,.T.);
#57994=EDGE_CURVE('',#41033,#43868,#35691,.T.);
#57995=EDGE_CURVE('',#43857,#40769,#35692,.T.);
#57996=EDGE_CURVE('',#41034,#43849,#35693,.T.);
#57997=EDGE_CURVE('',#43858,#41331,#35694,.T.);
#57998=EDGE_CURVE('',#41035,#43852,#35695,.T.);
#57999=EDGE_CURVE('',#43859,#41327,#2472,.T.);
#58000=EDGE_CURVE('',#41036,#43855,#35696,.T.);
#58001=EDGE_CURVE('',#43860,#41326,#35697,.T.);
#58002=EDGE_CURVE('',#41037,#43854,#35698,.T.);
#58003=EDGE_CURVE('',#43861,#41323,#35699,.T.);
#58004=EDGE_CURVE('',#41314,#43853,#35700,.T.);
#58005=EDGE_CURVE('',#43862,#41322,#35701,.T.);
#58006=EDGE_CURVE('',#41315,#43864,#2473,.T.);
#58007=EDGE_CURVE('',#43863,#41319,#35702,.T.);
#58008=EDGE_CURVE('',#43904,#41290,#2474,.T.);
#58009=EDGE_CURVE('',#41285,#43903,#35703,.T.);
#58010=EDGE_CURVE('',#41284,#43902,#35704,.T.);
#58011=EDGE_CURVE('',#43893,#41292,#35705,.T.);
#58012=EDGE_CURVE('',#41281,#43901,#35706,.T.);
#58013=EDGE_CURVE('',#43894,#40780,#35707,.T.);
#58014=EDGE_CURVE('',#41280,#43900,#35708,.T.);
#58015=EDGE_CURVE('',#43895,#40779,#35709,.T.);
#58016=EDGE_CURVE('',#41278,#43899,#2475,.T.);
#58017=EDGE_CURVE('',#43878,#40778,#35710,.T.);
#58018=EDGE_CURVE('',#41273,#43898,#35711,.T.);
#58019=EDGE_CURVE('',#43879,#40777,#35712,.T.);
#58020=EDGE_CURVE('',#41026,#43897,#35713,.T.);
#58021=EDGE_CURVE('',#43884,#40776,#35714,.T.);
#58022=EDGE_CURVE('',#41027,#43896,#35715,.T.);
#58023=EDGE_CURVE('',#43885,#40775,#35716,.T.);
#58024=EDGE_CURVE('',#41028,#43877,#35717,.T.);
#58025=EDGE_CURVE('',#43886,#41311,#35718,.T.);
#58026=EDGE_CURVE('',#41029,#43880,#35719,.T.);
#58027=EDGE_CURVE('',#43887,#41307,#2476,.T.);
#58028=EDGE_CURVE('',#41030,#43883,#35720,.T.);
#58029=EDGE_CURVE('',#43888,#41306,#35721,.T.);
#58030=EDGE_CURVE('',#41031,#43882,#35722,.T.);
#58031=EDGE_CURVE('',#43889,#41303,#35723,.T.);
#58032=EDGE_CURVE('',#41294,#43881,#35724,.T.);
#58033=EDGE_CURVE('',#43890,#41302,#35725,.T.);
#58034=EDGE_CURVE('',#41295,#43892,#2477,.T.);
#58035=EDGE_CURVE('',#43891,#41299,#35726,.T.);
#58036=EDGE_CURVE('',#43932,#41270,#2478,.T.);
#58037=EDGE_CURVE('',#41265,#43931,#35727,.T.);
#58038=EDGE_CURVE('',#41264,#43930,#35728,.T.);
#58039=EDGE_CURVE('',#43921,#41272,#35729,.T.);
#58040=EDGE_CURVE('',#41261,#43929,#35730,.T.);
#58041=EDGE_CURVE('',#43922,#40786,#35731,.T.);
#58042=EDGE_CURVE('',#41260,#43928,#35732,.T.);
#58043=EDGE_CURVE('',#43923,#40785,#35733,.T.);
#58044=EDGE_CURVE('',#41258,#43927,#2479,.T.);
#58045=EDGE_CURVE('',#43906,#40784,#35734,.T.);
#58046=EDGE_CURVE('',#41253,#43926,#35735,.T.);
#58047=EDGE_CURVE('',#43907,#40783,#35736,.T.);
#58048=EDGE_CURVE('',#41020,#43925,#35737,.T.);
#58049=EDGE_CURVE('',#43912,#40782,#35738,.T.);
#58050=EDGE_CURVE('',#41021,#43924,#35739,.T.);
#58051=EDGE_CURVE('',#43913,#40781,#35740,.T.);
#58052=EDGE_CURVE('',#41022,#43905,#35741,.T.);
#58053=EDGE_CURVE('',#43914,#41291,#35742,.T.);
#58054=EDGE_CURVE('',#41023,#43908,#35743,.T.);
#58055=EDGE_CURVE('',#43915,#41287,#2480,.T.);
#58056=EDGE_CURVE('',#41024,#43911,#35744,.T.);
#58057=EDGE_CURVE('',#43916,#41286,#35745,.T.);
#58058=EDGE_CURVE('',#41025,#43910,#35746,.T.);
#58059=EDGE_CURVE('',#43917,#41283,#35747,.T.);
#58060=EDGE_CURVE('',#41274,#43909,#35748,.T.);
#58061=EDGE_CURVE('',#43918,#41282,#35749,.T.);
#58062=EDGE_CURVE('',#41275,#43920,#2481,.T.);
#58063=EDGE_CURVE('',#43919,#41279,#35750,.T.);
#58064=EDGE_CURVE('',#43960,#41250,#2482,.T.);
#58065=EDGE_CURVE('',#41245,#43959,#35751,.T.);
#58066=EDGE_CURVE('',#41244,#43958,#35752,.T.);
#58067=EDGE_CURVE('',#43949,#41252,#35753,.T.);
#58068=EDGE_CURVE('',#41241,#43957,#35754,.T.);
#58069=EDGE_CURVE('',#43950,#40792,#35755,.T.);
#58070=EDGE_CURVE('',#41240,#43956,#35756,.T.);
#58071=EDGE_CURVE('',#43951,#40791,#35757,.T.);
#58072=EDGE_CURVE('',#41238,#43955,#2483,.T.);
#58073=EDGE_CURVE('',#43934,#40790,#35758,.T.);
#58074=EDGE_CURVE('',#41233,#43954,#35759,.T.);
#58075=EDGE_CURVE('',#43935,#40789,#35760,.T.);
#58076=EDGE_CURVE('',#41014,#43953,#35761,.T.);
#58077=EDGE_CURVE('',#43940,#40788,#35762,.T.);
#58078=EDGE_CURVE('',#41015,#43952,#35763,.T.);
#58079=EDGE_CURVE('',#43941,#40787,#35764,.T.);
#58080=EDGE_CURVE('',#41016,#43933,#35765,.T.);
#58081=EDGE_CURVE('',#43942,#41271,#35766,.T.);
#58082=EDGE_CURVE('',#41017,#43936,#35767,.T.);
#58083=EDGE_CURVE('',#43943,#41267,#2484,.T.);
#58084=EDGE_CURVE('',#41018,#43939,#35768,.T.);
#58085=EDGE_CURVE('',#43944,#41266,#35769,.T.);
#58086=EDGE_CURVE('',#41019,#43938,#35770,.T.);
#58087=EDGE_CURVE('',#43945,#41263,#35771,.T.);
#58088=EDGE_CURVE('',#41254,#43937,#35772,.T.);
#58089=EDGE_CURVE('',#43946,#41262,#35773,.T.);
#58090=EDGE_CURVE('',#41255,#43948,#2485,.T.);
#58091=EDGE_CURVE('',#43947,#41259,#35774,.T.);
#58092=EDGE_CURVE('',#43988,#41230,#2486,.T.);
#58093=EDGE_CURVE('',#41225,#43987,#35775,.T.);
#58094=EDGE_CURVE('',#41224,#43986,#35776,.T.);
#58095=EDGE_CURVE('',#43977,#41232,#35777,.T.);
#58096=EDGE_CURVE('',#41221,#43985,#35778,.T.);
#58097=EDGE_CURVE('',#43978,#40798,#35779,.T.);
#58098=EDGE_CURVE('',#41220,#43984,#35780,.T.);
#58099=EDGE_CURVE('',#43979,#40797,#35781,.T.);
#58100=EDGE_CURVE('',#41218,#43983,#2487,.T.);
#58101=EDGE_CURVE('',#43962,#40796,#35782,.T.);
#58102=EDGE_CURVE('',#41213,#43982,#35783,.T.);
#58103=EDGE_CURVE('',#43963,#40795,#35784,.T.);
#58104=EDGE_CURVE('',#41008,#43981,#35785,.T.);
#58105=EDGE_CURVE('',#43968,#40794,#35786,.T.);
#58106=EDGE_CURVE('',#41009,#43980,#35787,.T.);
#58107=EDGE_CURVE('',#43969,#40793,#35788,.T.);
#58108=EDGE_CURVE('',#41010,#43961,#35789,.T.);
#58109=EDGE_CURVE('',#43970,#41251,#35790,.T.);
#58110=EDGE_CURVE('',#41011,#43964,#35791,.T.);
#58111=EDGE_CURVE('',#43971,#41247,#2488,.T.);
#58112=EDGE_CURVE('',#41012,#43967,#35792,.T.);
#58113=EDGE_CURVE('',#43972,#41246,#35793,.T.);
#58114=EDGE_CURVE('',#41013,#43966,#35794,.T.);
#58115=EDGE_CURVE('',#43973,#41243,#35795,.T.);
#58116=EDGE_CURVE('',#41234,#43965,#35796,.T.);
#58117=EDGE_CURVE('',#43974,#41242,#35797,.T.);
#58118=EDGE_CURVE('',#41235,#43976,#2489,.T.);
#58119=EDGE_CURVE('',#43975,#41239,#35798,.T.);
#58120=EDGE_CURVE('',#44016,#41210,#2490,.T.);
#58121=EDGE_CURVE('',#41205,#44015,#35799,.T.);
#58122=EDGE_CURVE('',#41204,#44014,#35800,.T.);
#58123=EDGE_CURVE('',#44005,#41212,#35801,.T.);
#58124=EDGE_CURVE('',#41201,#44013,#35802,.T.);
#58125=EDGE_CURVE('',#44006,#40804,#35803,.T.);
#58126=EDGE_CURVE('',#41200,#44012,#35804,.T.);
#58127=EDGE_CURVE('',#44007,#40803,#35805,.T.);
#58128=EDGE_CURVE('',#41198,#44011,#2491,.T.);
#58129=EDGE_CURVE('',#43990,#40802,#35806,.T.);
#58130=EDGE_CURVE('',#41193,#44010,#35807,.T.);
#58131=EDGE_CURVE('',#43991,#40801,#35808,.T.);
#58132=EDGE_CURVE('',#41002,#44009,#35809,.T.);
#58133=EDGE_CURVE('',#43996,#40800,#35810,.T.);
#58134=EDGE_CURVE('',#41003,#44008,#35811,.T.);
#58135=EDGE_CURVE('',#43997,#40799,#35812,.T.);
#58136=EDGE_CURVE('',#41004,#43989,#35813,.T.);
#58137=EDGE_CURVE('',#43998,#41231,#35814,.T.);
#58138=EDGE_CURVE('',#41005,#43992,#35815,.T.);
#58139=EDGE_CURVE('',#43999,#41227,#2492,.T.);
#58140=EDGE_CURVE('',#41006,#43995,#35816,.T.);
#58141=EDGE_CURVE('',#44000,#41226,#35817,.T.);
#58142=EDGE_CURVE('',#41007,#43994,#35818,.T.);
#58143=EDGE_CURVE('',#44001,#41223,#35819,.T.);
#58144=EDGE_CURVE('',#41214,#43993,#35820,.T.);
#58145=EDGE_CURVE('',#44002,#41222,#35821,.T.);
#58146=EDGE_CURVE('',#41215,#44004,#2493,.T.);
#58147=EDGE_CURVE('',#44003,#41219,#35822,.T.);
#58148=EDGE_CURVE('',#44044,#41185,#2494,.T.);
#58149=EDGE_CURVE('',#41187,#44043,#35823,.T.);
#58150=EDGE_CURVE('',#41182,#44042,#35824,.T.);
#58151=EDGE_CURVE('',#44033,#41192,#35825,.T.);
#58152=EDGE_CURVE('',#41183,#44041,#35826,.T.);
#58153=EDGE_CURVE('',#44034,#40810,#35827,.T.);
#58154=EDGE_CURVE('',#41180,#44040,#35828,.T.);
#58155=EDGE_CURVE('',#44035,#40809,#35829,.T.);
#58156=EDGE_CURVE('',#41173,#44039,#2495,.T.);
#58157=EDGE_CURVE('',#44018,#40808,#35830,.T.);
#58158=EDGE_CURVE('',#41175,#44038,#35831,.T.);
#58159=EDGE_CURVE('',#44019,#40807,#35832,.T.);
#58160=EDGE_CURVE('',#40996,#44037,#35833,.T.);
#58161=EDGE_CURVE('',#44024,#40806,#35834,.T.);
#58162=EDGE_CURVE('',#40997,#44036,#35835,.T.);
#58163=EDGE_CURVE('',#44025,#40805,#35836,.T.);
#58164=EDGE_CURVE('',#40998,#44017,#35837,.T.);
#58165=EDGE_CURVE('',#44026,#41211,#35838,.T.);
#58166=EDGE_CURVE('',#40999,#44020,#35839,.T.);
#58167=EDGE_CURVE('',#44027,#41207,#2496,.T.);
#58168=EDGE_CURVE('',#41000,#44023,#35840,.T.);
#58169=EDGE_CURVE('',#44028,#41206,#35841,.T.);
#58170=EDGE_CURVE('',#41001,#44022,#35842,.T.);
#58171=EDGE_CURVE('',#44029,#41203,#35843,.T.);
#58172=EDGE_CURVE('',#41194,#44021,#35844,.T.);
#58173=EDGE_CURVE('',#44030,#41202,#35845,.T.);
#58174=EDGE_CURVE('',#41195,#44032,#2497,.T.);
#58175=EDGE_CURVE('',#44031,#41199,#35846,.T.);
#58176=EDGE_CURVE('',#44045,#44045,#35847,.T.);
#58177=EDGE_CURVE('',#44045,#44046,#35848,.T.);
#58178=EDGE_CURVE('',#44046,#44046,#35849,.T.);
#58179=EDGE_CURVE('',#44047,#44047,#35850,.T.);
#58180=EDGE_CURVE('',#44047,#44048,#35851,.T.);
#58181=EDGE_CURVE('',#44048,#44048,#35852,.T.);
#58182=EDGE_CURVE('',#44049,#44049,#35853,.T.);
#58183=EDGE_CURVE('',#44049,#44050,#35854,.T.);
#58184=EDGE_CURVE('',#44051,#44050,#35855,.T.);
#58185=EDGE_CURVE('',#44050,#44051,#35856,.T.);
#58186=EDGE_CURVE('',#44052,#44052,#35857,.T.);
#58187=EDGE_CURVE('',#44052,#44045,#23960,.T.);
#58188=EDGE_CURVE('',#44048,#44051,#23961,.T.);
#58189=EDGE_CURVE('',#44053,#44053,#35858,.T.);
#58190=EDGE_CURVE('',#44053,#44054,#23962,.T.);
#58191=EDGE_CURVE('',#44054,#44054,#35859,.T.);
#58192=EDGE_CURVE('',#44055,#44055,#35860,.T.);
#58193=EDGE_CURVE('',#44055,#44056,#35861,.T.);
#58194=EDGE_CURVE('',#44056,#44056,#35862,.T.);
#58195=EDGE_CURVE('',#44057,#44057,#35863,.T.);
#58196=EDGE_CURVE('',#44057,#44058,#35864,.T.);
#58197=EDGE_CURVE('',#44058,#44058,#35865,.T.);
#58198=EDGE_CURVE('',#44059,#44059,#35866,.T.);
#58199=EDGE_CURVE('',#44059,#44055,#23963,.T.);
#58200=EDGE_CURVE('',#44058,#44060,#23964,.T.);
#58201=EDGE_CURVE('',#44060,#44060,#35867,.T.);
#58202=EDGE_CURVE('',#44061,#44061,#35868,.T.);
#58203=EDGE_CURVE('',#44061,#44062,#35869,.T.);
#58204=EDGE_CURVE('',#44062,#44062,#35870,.T.);
#58205=EDGE_CURVE('',#44063,#44064,#35871,.T.);
#58206=EDGE_CURVE('',#44065,#44063,#35872,.T.);
#58207=EDGE_CURVE('',#44066,#44065,#35873,.T.);
#58208=EDGE_CURVE('',#44066,#44064,#35874,.T.);
#58209=EDGE_CURVE('',#44067,#44068,#35875,.T.);
#58210=EDGE_CURVE('',#44067,#44069,#35876,.T.);
#58211=EDGE_CURVE('',#44070,#44069,#35877,.T.);
#58212=EDGE_CURVE('',#44068,#44070,#35878,.T.);
#58213=EDGE_CURVE('',#44071,#44072,#35879,.T.);
#58214=EDGE_CURVE('',#44071,#44073,#35880,.T.);
#58215=EDGE_CURVE('',#44074,#44073,#35881,.T.);
#58216=EDGE_CURVE('',#44072,#44074,#35882,.T.);
#58217=EDGE_CURVE('',#44075,#44076,#35883,.T.);
#58218=EDGE_CURVE('',#44075,#44077,#35884,.T.);
#58219=EDGE_CURVE('',#44078,#44077,#35885,.T.);
#58220=EDGE_CURVE('',#44076,#44078,#35886,.T.);
#58221=EDGE_CURVE('',#44079,#44080,#35887,.T.);
#58222=EDGE_CURVE('',#44081,#44079,#35888,.T.);
#58223=EDGE_CURVE('',#44082,#44081,#35889,.T.);
#58224=EDGE_CURVE('',#44080,#44082,#35890,.T.);
#58225=EDGE_CURVE('',#44083,#44084,#35891,.T.);
#58226=EDGE_CURVE('',#44083,#44085,#35892,.T.);
#58227=EDGE_CURVE('',#44086,#44085,#35893,.T.);
#58228=EDGE_CURVE('',#44084,#44086,#35894,.T.);
#58229=EDGE_CURVE('',#44085,#44087,#35895,.T.);
#58230=EDGE_CURVE('',#44088,#44083,#35896,.T.);
#58231=EDGE_CURVE('',#44088,#44087,#35897,.T.);
#58232=EDGE_CURVE('',#44089,#44088,#35898,.T.);
#58233=EDGE_CURVE('',#44090,#44089,#35899,.T.);
#58234=EDGE_CURVE('',#44087,#44090,#35900,.T.);
#58235=EDGE_CURVE('',#44091,#44077,#23965,.T.);
#58236=EDGE_CURVE('',#44092,#44091,#35901,.T.);
#58237=EDGE_CURVE('',#44092,#44093,#5215,.T.);
#58238=EDGE_CURVE('',#44093,#44094,#5216,.T.);
#58239=EDGE_CURVE('',#44078,#44094,#23966,.T.);
#58240=EDGE_CURVE('',#44095,#44081,#23967,.T.);
#58241=EDGE_CURVE('',#44095,#44096,#5217,.T.);
#58242=EDGE_CURVE('',#44096,#44097,#5218,.T.);
#58243=EDGE_CURVE('',#44098,#44097,#35902,.T.);
#58244=EDGE_CURVE('',#44082,#44098,#23968,.T.);
#58245=EDGE_CURVE('',#44099,#44100,#35903,.T.);
#58246=EDGE_CURVE('',#44099,#44091,#5219,.T.);
#58247=EDGE_CURVE('',#44098,#44091,#35904,.T.);
#58248=EDGE_CURVE('',#44098,#44100,#5220,.T.);
#58249=EDGE_CURVE('',#44101,#44101,#35905,.T.);
#58250=EDGE_CURVE('',#44101,#44102,#23969,.T.);
#58251=EDGE_CURVE('',#44102,#44102,#35906,.T.);
#58252=EDGE_CURVE('',#44103,#44103,#35907,.T.);
#58253=EDGE_CURVE('',#44103,#44104,#23970,.T.);
#58254=EDGE_CURVE('',#44104,#44104,#35908,.T.);
#58255=EDGE_CURVE('',#44105,#44105,#35909,.T.);
#58256=EDGE_CURVE('',#44105,#44106,#23971,.T.);
#58257=EDGE_CURVE('',#44106,#44106,#35910,.T.);
#58258=EDGE_CURVE('',#44107,#44107,#35911,.T.);
#58259=EDGE_CURVE('',#44107,#44108,#23972,.T.);
#58260=EDGE_CURVE('',#44108,#44108,#35912,.T.);
#58261=EDGE_CURVE('',#44109,#44109,#35913,.T.);
#58262=EDGE_CURVE('',#44109,#44110,#23973,.T.);
#58263=EDGE_CURVE('',#44110,#44110,#35914,.T.);
#58264=EDGE_CURVE('',#44087,#44111,#23974,.T.);
#58265=EDGE_CURVE('',#44111,#44112,#35915,.T.);
#58266=EDGE_CURVE('',#44112,#44085,#23975,.T.);
#58267=EDGE_CURVE('',#44064,#44113,#5221,.T.);
#58268=EDGE_CURVE('',#44113,#44114,#35916,.T.);
#58269=EDGE_CURVE('',#44114,#44115,#5222,.T.);
#58270=EDGE_CURVE('',#44115,#44116,#5223,.T.);
#58271=EDGE_CURVE('',#44116,#44117,#35917,.T.);
#58272=EDGE_CURVE('',#44117,#44118,#5224,.T.);
#58273=EDGE_CURVE('',#44118,#44099,#5225,.T.);
#58274=EDGE_CURVE('',#44100,#44119,#5226,.T.);
#58275=EDGE_CURVE('',#44119,#44120,#5227,.T.);
#58276=EDGE_CURVE('',#44120,#44121,#35918,.T.);
#58277=EDGE_CURVE('',#44121,#44122,#5228,.T.);
#58278=EDGE_CURVE('',#44122,#44123,#5229,.T.);
#58279=EDGE_CURVE('',#44123,#44124,#35919,.T.);
#58280=EDGE_CURVE('',#44124,#44125,#5230,.T.);
#58281=EDGE_CURVE('',#44125,#44126,#5231,.T.);
#58282=EDGE_CURVE('',#44126,#44127,#35920,.T.);
#58283=EDGE_CURVE('',#44127,#44128,#5232,.T.);
#58284=EDGE_CURVE('',#44128,#44129,#5233,.T.);
#58285=EDGE_CURVE('',#44129,#44130,#35921,.T.);
#58286=EDGE_CURVE('',#44130,#44131,#5234,.T.);
#58287=EDGE_CURVE('',#44131,#44132,#5235,.T.);
#58288=EDGE_CURVE('',#44132,#44133,#35922,.T.);
#58289=EDGE_CURVE('',#44133,#44134,#5236,.T.);
#58290=EDGE_CURVE('',#44134,#44135,#5237,.T.);
#58291=EDGE_CURVE('',#44135,#44136,#35923,.T.);
#58292=EDGE_CURVE('',#44136,#44063,#5238,.T.);
#58293=EDGE_CURVE('',#44137,#44138,#35924,.T.);
#58294=EDGE_CURVE('',#44139,#44138,#23976,.T.);
#58295=EDGE_CURVE('',#44139,#44140,#35925,.T.);
#58296=EDGE_CURVE('',#44140,#44141,#5239,.T.);
#58297=EDGE_CURVE('',#44141,#44142,#23977,.T.);
#58298=EDGE_CURVE('',#44143,#44142,#35926,.T.);
#58299=EDGE_CURVE('',#44144,#44143,#23978,.T.);
#58300=EDGE_CURVE('',#44144,#44145,#5240,.T.);
#58301=EDGE_CURVE('',#44145,#44146,#35927,.T.);
#58302=EDGE_CURVE('',#44146,#44137,#23979,.T.);
#58303=EDGE_CURVE('',#44147,#44148,#35928,.T.);
#58304=EDGE_CURVE('',#44149,#44148,#23980,.T.);
#58305=EDGE_CURVE('',#44149,#44150,#35929,.T.);
#58306=EDGE_CURVE('',#44150,#44151,#5241,.T.);
#58307=EDGE_CURVE('',#44151,#44152,#23981,.T.);
#58308=EDGE_CURVE('',#44153,#44152,#35930,.T.);
#58309=EDGE_CURVE('',#44154,#44153,#23982,.T.);
#58310=EDGE_CURVE('',#44154,#44155,#5242,.T.);
#58311=EDGE_CURVE('',#44155,#44156,#35931,.T.);
#58312=EDGE_CURVE('',#44156,#44147,#23983,.T.);
#58313=EDGE_CURVE('',#44157,#44158,#23984,.T.);
#58314=EDGE_CURVE('',#44157,#44154,#23985,.T.);
#58315=EDGE_CURVE('',#44158,#44153,#23986,.T.);
#58316=EDGE_CURVE('',#44151,#44144,#23987,.T.);
#58317=EDGE_CURVE('',#44152,#44143,#23988,.T.);
#58318=EDGE_CURVE('',#44159,#44160,#23989,.T.);
#58319=EDGE_CURVE('',#44159,#44161,#23990,.T.);
#58320=EDGE_CURVE('',#44161,#44162,#23991,.T.);
#58321=EDGE_CURVE('',#44160,#44162,#23992,.T.);
#58322=EDGE_CURVE('',#44163,#44067,#23993,.T.);
#58323=EDGE_CURVE('',#44164,#44068,#23994,.T.);
#58324=EDGE_CURVE('',#44164,#44165,#35932,.T.);
#58325=EDGE_CURVE('',#44165,#44157,#5243,.T.);
#58326=EDGE_CURVE('',#44162,#44158,#35933,.T.);
#58327=EDGE_CURVE('',#44161,#44166,#5244,.T.);
#58328=EDGE_CURVE('',#44166,#44163,#35934,.T.);
#58329=EDGE_CURVE('',#44167,#44071,#23995,.T.);
#58330=EDGE_CURVE('',#44168,#44072,#23996,.T.);
#58331=EDGE_CURVE('',#44168,#44169,#35935,.T.);
#58332=EDGE_CURVE('',#44169,#44159,#5245,.T.);
#58333=EDGE_CURVE('',#44170,#44160,#35936,.T.);
#58334=EDGE_CURVE('',#44171,#44170,#23997,.T.);
#58335=EDGE_CURVE('',#44171,#44172,#5246,.T.);
#58336=EDGE_CURVE('',#44172,#44167,#35937,.T.);
#58337=EDGE_CURVE('',#44173,#44174,#5247,.T.);
#58338=EDGE_CURVE('',#44174,#44171,#23998,.T.);
#58339=EDGE_CURVE('',#44142,#44170,#23999,.T.);
#58340=EDGE_CURVE('',#44141,#44173,#24000,.T.);
#58341=EDGE_CURVE('',#44175,#44176,#24001,.T.);
#58342=EDGE_CURVE('',#44175,#44177,#35938,.T.);
#58343=EDGE_CURVE('',#44177,#44178,#24002,.T.);
#58344=EDGE_CURVE('',#44176,#44178,#35939,.T.);
#58345=EDGE_CURVE('',#44177,#44179,#24003,.T.);
#58346=EDGE_CURVE('',#44179,#44180,#24004,.T.);
#58347=EDGE_CURVE('',#44178,#44180,#24005,.T.);
#58348=EDGE_CURVE('',#44179,#44181,#35940,.T.);
#58349=EDGE_CURVE('',#44181,#44182,#24006,.T.);
#58350=EDGE_CURVE('',#44180,#44182,#35941,.T.);
#58351=EDGE_CURVE('',#44181,#44183,#24007,.T.);
#58352=EDGE_CURVE('',#44183,#44184,#24008,.T.);
#58353=EDGE_CURVE('',#44182,#44184,#24009,.T.);
#58354=EDGE_CURVE('',#44183,#44185,#35942,.T.);
#58355=EDGE_CURVE('',#44185,#44186,#24010,.T.);
#58356=EDGE_CURVE('',#44184,#44186,#35943,.T.);
#58357=EDGE_CURVE('',#44185,#44187,#24011,.T.);
#58358=EDGE_CURVE('',#44187,#44188,#24012,.T.);
#58359=EDGE_CURVE('',#44186,#44188,#24013,.T.);
#58360=EDGE_CURVE('',#44187,#44189,#35944,.T.);
#58361=EDGE_CURVE('',#44189,#44190,#24014,.T.);
#58362=EDGE_CURVE('',#44188,#44190,#35945,.T.);
#58363=EDGE_CURVE('',#44189,#44175,#24015,.T.);
#58364=EDGE_CURVE('',#44190,#44176,#24016,.T.);
#58365=EDGE_CURVE('',#44065,#44191,#5248,.T.);
#58366=EDGE_CURVE('',#44191,#44192,#24017,.T.);
#58367=EDGE_CURVE('',#44192,#44193,#35946,.T.);
#58368=EDGE_CURVE('',#44193,#44194,#24018,.T.);
#58369=EDGE_CURVE('',#44194,#44066,#5249,.T.);
#58370=EDGE_CURVE('',#44195,#44196,#5250,.T.);
#58371=EDGE_CURVE('',#44196,#44197,#24019,.T.);
#58372=EDGE_CURVE('',#44198,#44197,#24020,.T.);
#58373=EDGE_CURVE('',#44198,#44199,#5251,.T.);
#58374=EDGE_CURVE('',#44199,#44200,#5252,.T.);
#58375=EDGE_CURVE('',#44200,#44201,#5253,.T.);
#58376=EDGE_CURVE('',#44201,#44202,#24021,.T.);
#58377=EDGE_CURVE('',#44202,#44195,#35947,.T.);
#58378=EDGE_CURVE('',#44203,#44204,#24022,.T.);
#58379=EDGE_CURVE('',#44204,#44205,#24023,.T.);
#58380=EDGE_CURVE('',#44205,#44206,#5254,.T.);
#58381=EDGE_CURVE('',#44206,#44207,#35948,.T.);
#58382=EDGE_CURVE('',#44207,#44208,#24024,.T.);
#58383=EDGE_CURVE('',#44208,#44209,#5255,.T.);
#58384=EDGE_CURVE('',#44209,#44210,#5256,.T.);
#58385=EDGE_CURVE('',#44210,#44203,#5257,.T.);
#58386=EDGE_CURVE('',#44197,#44204,#35949,.T.);
#58387=EDGE_CURVE('',#44203,#44198,#5258,.T.);
#58388=EDGE_CURVE('',#44199,#44210,#5259,.T.);
#58389=EDGE_CURVE('',#44209,#44211,#5260,.T.);
#58390=EDGE_CURVE('',#44211,#44212,#5261,.T.);
#58391=EDGE_CURVE('',#44212,#44200,#5262,.T.);
#58392=EDGE_CURVE('',#44213,#44214,#35950,.T.);
#58393=EDGE_CURVE('',#44214,#44215,#24025,.T.);
#58394=EDGE_CURVE('',#44215,#44216,#35951,.T.);
#58395=EDGE_CURVE('',#44216,#44213,#24026,.T.);
#58396=EDGE_CURVE('',#44172,#44217,#24027,.T.);
#58397=EDGE_CURVE('',#44217,#44218,#5263,.T.);
#58398=EDGE_CURVE('',#44218,#44214,#35952,.T.);
#58399=EDGE_CURVE('',#44213,#44219,#35953,.T.);
#58400=EDGE_CURVE('',#44167,#44219,#24028,.T.);
#58401=EDGE_CURVE('',#44220,#44221,#35954,.T.);
#58402=EDGE_CURVE('',#44221,#44222,#5264,.T.);
#58403=EDGE_CURVE('',#44222,#44140,#24029,.T.);
#58404=EDGE_CURVE('',#44223,#44139,#24030,.T.);
#58405=EDGE_CURVE('',#44223,#44224,#35955,.T.);
#58406=EDGE_CURVE('',#44220,#44224,#35956,.T.);
#58407=EDGE_CURVE('',#44225,#44226,#35957,.T.);
#58408=EDGE_CURVE('',#44226,#44220,#24031,.T.);
#58409=EDGE_CURVE('',#44224,#44225,#24032,.T.);
#58410=EDGE_CURVE('',#44227,#44228,#24033,.T.);
#58411=EDGE_CURVE('',#44228,#44229,#35958,.T.);
#58412=EDGE_CURVE('',#44229,#44230,#24034,.T.);
#58413=EDGE_CURVE('',#44230,#44227,#35959,.T.);
#58414=EDGE_CURVE('',#44077,#44082,#35960,.T.);
#58415=EDGE_CURVE('',#44231,#44232,#24035,.T.);
#58416=EDGE_CURVE('',#44232,#44233,#35961,.T.);
#58417=EDGE_CURVE('',#44233,#44234,#24036,.T.);
#58418=EDGE_CURVE('',#44234,#44231,#35962,.T.);
#58419=EDGE_CURVE('',#44235,#44236,#24037,.T.);
#58420=EDGE_CURVE('',#44236,#44237,#35963,.T.);
#58421=EDGE_CURVE('',#44237,#44238,#24038,.T.);
#58422=EDGE_CURVE('',#44238,#44235,#35964,.T.);
#58423=EDGE_CURVE('',#44069,#44239,#24039,.T.);
#58424=EDGE_CURVE('',#44239,#44240,#35965,.T.);
#58425=EDGE_CURVE('',#44240,#44070,#24040,.T.);
#58426=EDGE_CURVE('',#44073,#44241,#24041,.T.);
#58427=EDGE_CURVE('',#44241,#44242,#35966,.T.);
#58428=EDGE_CURVE('',#44242,#44074,#24042,.T.);
#58429=EDGE_CURVE('',#44219,#44243,#24043,.T.);
#58430=EDGE_CURVE('',#44243,#44244,#5265,.T.);
#58431=EDGE_CURVE('',#44244,#44245,#5266,.T.);
#58432=EDGE_CURVE('',#44245,#44071,#24044,.T.);
#58433=EDGE_CURVE('',#44138,#44246,#24045,.T.);
#58434=EDGE_CURVE('',#44246,#44247,#5267,.T.);
#58435=EDGE_CURVE('',#44247,#44248,#5268,.T.);
#58436=EDGE_CURVE('',#44248,#44223,#24046,.T.);
#58437=EDGE_CURVE('',#44094,#44249,#5269,.T.);
#58438=EDGE_CURVE('',#44249,#44250,#5270,.T.);
#58439=EDGE_CURVE('',#44250,#44137,#24047,.T.);
#58440=EDGE_CURVE('',#44146,#44078,#24048,.T.);
#58441=EDGE_CURVE('',#44251,#44252,#35967,.T.);
#58442=EDGE_CURVE('',#44252,#44253,#24049,.T.);
#58443=EDGE_CURVE('',#44253,#44254,#35968,.T.);
#58444=EDGE_CURVE('',#44254,#44079,#24050,.T.);
#58445=EDGE_CURVE('',#44080,#44075,#35969,.T.);
#58446=EDGE_CURVE('',#44076,#44251,#24051,.T.);
#58447=EDGE_CURVE('',#44148,#44255,#24052,.T.);
#58448=EDGE_CURVE('',#44255,#44256,#5271,.T.);
#58449=EDGE_CURVE('',#44256,#44095,#5272,.T.);
#58450=EDGE_CURVE('',#44081,#44149,#24053,.T.);
#58451=EDGE_CURVE('',#44257,#44258,#24054,.T.);
#58452=EDGE_CURVE('',#44258,#44259,#5273,.T.);
#58453=EDGE_CURVE('',#44259,#44260,#5274,.T.);
#58454=EDGE_CURVE('',#44260,#44147,#24055,.T.);
#58455=EDGE_CURVE('',#44156,#44257,#24056,.T.);
#58456=EDGE_CURVE('',#44261,#44262,#35970,.T.);
#58457=EDGE_CURVE('',#44262,#44263,#24057,.T.);
#58458=EDGE_CURVE('',#44263,#44264,#35971,.T.);
#58459=EDGE_CURVE('',#44264,#44265,#24058,.T.);
#58460=EDGE_CURVE('',#44265,#44266,#35972,.T.);
#58461=EDGE_CURVE('',#44266,#44267,#35973,.T.);
#58462=EDGE_CURVE('',#44267,#44268,#35974,.T.);
#58463=EDGE_CURVE('',#44268,#44261,#24059,.T.);
#58464=EDGE_CURVE('',#44068,#44269,#24060,.T.);
#58465=EDGE_CURVE('',#44269,#44270,#5275,.T.);
#58466=EDGE_CURVE('',#44270,#44271,#5276,.T.);
#58467=EDGE_CURVE('',#44271,#44272,#24061,.T.);
#58468=EDGE_CURVE('',#44272,#44164,#24062,.T.);
#58469=EDGE_CURVE('',#44086,#44273,#24063,.T.);
#58470=EDGE_CURVE('',#44273,#44274,#5277,.T.);
#58471=EDGE_CURVE('',#44274,#44275,#5278,.T.);
#58472=EDGE_CURVE('',#44275,#44067,#24064,.T.);
#58473=EDGE_CURVE('',#44163,#44086,#24065,.T.);
#58474=EDGE_CURVE('',#44276,#44277,#35975,.T.);
#58475=EDGE_CURVE('',#44277,#44278,#24066,.T.);
#58476=EDGE_CURVE('',#44278,#44279,#35976,.T.);
#58477=EDGE_CURVE('',#44279,#44089,#24067,.T.);
#58478=EDGE_CURVE('',#44084,#44276,#24068,.T.);
#58479=EDGE_CURVE('',#44072,#44280,#24069,.T.);
#58480=EDGE_CURVE('',#44280,#44281,#2498,.T.);
#58481=EDGE_CURVE('',#44281,#44090,#24070,.T.);
#58482=EDGE_CURVE('',#44090,#44168,#24071,.T.);
#58483=EDGE_CURVE('',#44215,#44136,#35977,.T.);
#58484=EDGE_CURVE('',#44135,#44216,#5279,.T.);
#58485=EDGE_CURVE('',#44113,#44226,#35978,.T.);
#58486=EDGE_CURVE('',#44225,#44114,#5280,.T.);
#58487=EDGE_CURVE('',#44123,#44235,#5281,.T.);
#58488=EDGE_CURVE('',#44238,#44124,#5282,.T.);
#58489=EDGE_CURVE('',#44129,#44112,#5283,.T.);
#58490=EDGE_CURVE('',#44111,#44130,#5284,.T.);
#58491=EDGE_CURVE('',#44282,#44235,#35979,.T.);
#58492=EDGE_CURVE('',#44282,#44258,#5285,.T.);
#58493=EDGE_CURVE('',#44257,#44236,#35980,.T.);
#58494=EDGE_CURVE('',#44123,#44283,#5286,.T.);
#58495=EDGE_CURVE('',#44283,#44282,#5287,.T.);
#58496=EDGE_CURVE('',#44271,#44284,#5288,.T.);
#58497=EDGE_CURVE('',#44238,#44284,#35981,.T.);
#58498=EDGE_CURVE('',#44237,#44272,#35982,.T.);
#58499=EDGE_CURVE('',#44284,#44285,#5289,.T.);
#58500=EDGE_CURVE('',#44285,#44124,#5290,.T.);
#58501=EDGE_CURVE('',#44286,#44112,#35983,.T.);
#58502=EDGE_CURVE('',#44286,#44273,#5291,.T.);
#58503=EDGE_CURVE('',#44129,#44287,#5292,.T.);
#58504=EDGE_CURVE('',#44287,#44286,#5293,.T.);
#58505=EDGE_CURVE('',#44281,#44288,#5294,.T.);
#58506=EDGE_CURVE('',#44288,#44289,#5295,.T.);
#58507=EDGE_CURVE('',#44111,#44289,#35984,.T.);
#58508=EDGE_CURVE('',#44289,#44290,#5296,.T.);
#58509=EDGE_CURVE('',#44290,#44130,#5297,.T.);
#58510=EDGE_CURVE('',#44291,#44216,#35985,.T.);
#58511=EDGE_CURVE('',#44291,#44243,#5298,.T.);
#58512=EDGE_CURVE('',#44135,#44292,#5299,.T.);
#58513=EDGE_CURVE('',#44292,#44291,#5300,.T.);
#58514=EDGE_CURVE('',#44248,#44293,#5301,.T.);
#58515=EDGE_CURVE('',#44225,#44293,#35986,.T.);
#58516=EDGE_CURVE('',#44293,#44294,#5302,.T.);
#58517=EDGE_CURVE('',#44294,#44114,#5303,.T.);
#58518=EDGE_CURVE('',#44097,#44295,#5304,.T.);
#58519=EDGE_CURVE('',#44295,#44100,#5305,.T.);
#58520=EDGE_CURVE('',#44099,#44296,#5306,.T.);
#58521=EDGE_CURVE('',#44296,#44092,#5307,.T.);
#58522=EDGE_CURVE('',#44266,#44237,#35987,.T.);
#58523=EDGE_CURVE('',#44272,#44265,#35988,.T.);
#58524=EDGE_CURVE('',#44164,#44264,#35989,.T.);
#58525=EDGE_CURVE('',#44267,#44236,#35990,.T.);
#58526=EDGE_CURVE('',#44165,#44263,#35991,.T.);
#58527=EDGE_CURVE('',#44268,#44257,#35992,.T.);
#58528=EDGE_CURVE('',#44157,#44263,#5308,.T.);
#58529=EDGE_CURVE('',#44261,#44156,#35993,.T.);
#58530=EDGE_CURVE('',#44154,#44262,#5309,.T.);
#58531=EDGE_CURVE('',#44262,#44155,#35994,.T.);
#58532=EDGE_CURVE('',#44168,#44279,#35995,.T.);
#58533=EDGE_CURVE('',#44169,#44278,#35996,.T.);
#58534=EDGE_CURVE('',#44159,#44278,#5310,.T.);
#58535=EDGE_CURVE('',#44276,#44163,#35997,.T.);
#58536=EDGE_CURVE('',#44161,#44277,#5311,.T.);
#58537=EDGE_CURVE('',#44277,#44166,#35998,.T.);
#58538=EDGE_CURVE('',#44149,#44254,#35999,.T.);
#58539=EDGE_CURVE('',#44150,#44253,#36000,.T.);
#58540=EDGE_CURVE('',#44151,#44253,#5312,.T.);
#58541=EDGE_CURVE('',#44251,#44146,#36001,.T.);
#58542=EDGE_CURVE('',#44144,#44252,#5313,.T.);
#58543=EDGE_CURVE('',#44252,#44145,#36002,.T.);
#58544=EDGE_CURVE('',#44222,#44173,#36003,.T.);
#58545=EDGE_CURVE('',#44211,#44174,#36004,.T.);
#58546=EDGE_CURVE('',#44173,#44212,#36005,.T.);
#58547=EDGE_CURVE('',#44174,#44217,#36006,.T.);
#58548=EDGE_CURVE('',#44250,#44228,#5314,.T.);
#58549=EDGE_CURVE('',#44137,#44227,#36007,.T.);
#58550=EDGE_CURVE('',#44138,#44230,#36008,.T.);
#58551=EDGE_CURVE('',#44229,#44246,#5315,.T.);
#58552=EDGE_CURVE('',#44245,#44241,#5316,.T.);
#58553=EDGE_CURVE('',#44242,#44280,#5317,.T.);
#58554=EDGE_CURVE('',#44275,#44239,#5318,.T.);
#58555=EDGE_CURVE('',#44240,#44269,#5319,.T.);
#58556=EDGE_CURVE('',#44260,#44232,#5320,.T.);
#58557=EDGE_CURVE('',#44147,#44231,#36009,.T.);
#58558=EDGE_CURVE('',#44148,#44234,#36010,.T.);
#58559=EDGE_CURVE('',#44233,#44255,#5321,.T.);
#58560=EDGE_CURVE('',#44259,#44297,#5322,.T.);
#58561=EDGE_CURVE('',#44297,#44122,#5323,.T.);
#58562=EDGE_CURVE('',#44232,#44121,#36011,.T.);
#58563=EDGE_CURVE('',#44233,#44120,#36012,.T.);
#58564=EDGE_CURVE('',#44119,#44298,#5324,.T.);
#58565=EDGE_CURVE('',#44298,#44256,#5325,.T.);
#58566=EDGE_CURVE('',#44274,#44299,#5326,.T.);
#58567=EDGE_CURVE('',#44299,#44128,#5327,.T.);
#58568=EDGE_CURVE('',#44239,#44127,#36013,.T.);
#58569=EDGE_CURVE('',#44240,#44126,#36014,.T.);
#58570=EDGE_CURVE('',#44125,#44300,#5328,.T.);
#58571=EDGE_CURVE('',#44300,#44270,#5329,.T.);
#58572=EDGE_CURVE('',#44244,#44301,#5330,.T.);
#58573=EDGE_CURVE('',#44301,#44134,#5331,.T.);
#58574=EDGE_CURVE('',#44241,#44133,#36015,.T.);
#58575=EDGE_CURVE('',#44242,#44132,#36016,.T.);
#58576=EDGE_CURVE('',#44131,#44302,#5332,.T.);
#58577=EDGE_CURVE('',#44302,#44303,#5333,.T.);
#58578=EDGE_CURVE('',#44303,#44280,#2499,.T.);
#58579=EDGE_CURVE('',#44115,#44304,#5334,.T.);
#58580=EDGE_CURVE('',#44304,#44247,#5335,.T.);
#58581=EDGE_CURVE('',#44116,#44229,#36017,.T.);
#58582=EDGE_CURVE('',#44117,#44228,#36018,.T.);
#58583=EDGE_CURVE('',#44249,#44305,#5336,.T.);
#58584=EDGE_CURVE('',#44305,#44118,#5337,.T.);
#58585=EDGE_CURVE('',#44205,#44063,#5338,.T.);
#58586=EDGE_CURVE('',#44206,#44136,#36019,.T.);
#58587=EDGE_CURVE('',#44207,#44215,#36020,.T.);
#58588=EDGE_CURVE('',#44218,#44208,#5339,.T.);
#58589=EDGE_CURVE('',#44064,#44196,#5340,.T.);
#58590=EDGE_CURVE('',#44113,#44195,#36021,.T.);
#58591=EDGE_CURVE('',#44226,#44202,#36022,.T.);
#58592=EDGE_CURVE('',#44201,#44221,#5341,.T.);
#58593=EDGE_CURVE('',#44211,#44217,#36023,.T.);
#58594=EDGE_CURVE('',#44222,#44212,#36024,.T.);
#58595=EDGE_CURVE('',#44281,#44303,#5342,.T.);
#58596=EDGE_CURVE('',#44288,#44303,#36025,.T.);
#58597=EDGE_CURVE('',#44289,#44302,#36026,.T.);
#58598=EDGE_CURVE('',#44290,#44131,#36027,.T.);
#58599=EDGE_CURVE('',#44301,#44291,#36028,.T.);
#58600=EDGE_CURVE('',#44134,#44292,#36029,.T.);
#58601=EDGE_CURVE('',#44293,#44304,#36030,.T.);
#58602=EDGE_CURVE('',#44294,#44115,#36031,.T.);
#58603=EDGE_CURVE('',#44305,#44092,#36032,.T.);
#58604=EDGE_CURVE('',#44118,#44296,#36033,.T.);
#58605=EDGE_CURVE('',#44097,#44298,#36034,.T.);
#58606=EDGE_CURVE('',#44295,#44119,#36035,.T.);
#58607=EDGE_CURVE('',#44297,#44282,#36036,.T.);
#58608=EDGE_CURVE('',#44122,#44283,#36037,.T.);
#58609=EDGE_CURVE('',#44125,#44285,#36038,.T.);
#58610=EDGE_CURVE('',#44300,#44284,#36039,.T.);
#58611=EDGE_CURVE('',#44299,#44286,#36040,.T.);
#58612=EDGE_CURVE('',#44128,#44287,#36041,.T.);
#58613=EDGE_CURVE('',#44196,#44194,#36042,.T.);
#58614=EDGE_CURVE('',#44197,#44193,#5343,.T.);
#58615=EDGE_CURVE('',#44191,#44205,#36043,.T.);
#58616=EDGE_CURVE('',#44204,#44192,#5344,.T.);
#58617=EDGE_CURVE('',#44306,#44307,#36044,.T.);
#58618=EDGE_CURVE('',#44308,#44309,#36045,.T.);
#58619=EDGE_CURVE('',#44308,#44310,#36046,.T.);
#58620=EDGE_CURVE('',#44310,#44310,#36047,.T.);
#58621=EDGE_CURVE('',#44309,#44308,#36048,.T.);
#58622=EDGE_CURVE('',#44311,#44312,#36049,.T.);
#58623=EDGE_CURVE('',#44311,#44313,#36050,.T.);
#58624=EDGE_CURVE('',#44313,#44313,#36051,.T.);
#58625=EDGE_CURVE('',#44312,#44311,#36052,.T.);
#58626=EDGE_CURVE('',#44314,#44315,#5345,.T.);
#58627=EDGE_CURVE('',#44314,#44316,#36053,.T.);
#58628=EDGE_CURVE('',#44317,#44316,#5346,.T.);
#58629=EDGE_CURVE('',#44318,#44317,#36054,.T.);
#58630=EDGE_CURVE('',#44319,#44318,#36055,.T.);
#58631=EDGE_CURVE('',#44315,#44319,#5347,.T.);
#58632=EDGE_CURVE('',#44320,#44318,#5348,.T.);
#58633=EDGE_CURVE('',#44316,#44320,#5349,.T.);
#58634=EDGE_CURVE('',#44321,#44321,#36056,.T.);
#58635=EDGE_CURVE('',#44321,#44322,#24072,.T.);
#58636=EDGE_CURVE('',#44322,#44314,#36057,.T.);
#58637=EDGE_CURVE('',#44319,#44322,#5350,.T.);
#58638=EDGE_CURVE('',#44312,#44309,#24073,.T.);
#58639=EDGE_CURVE('',#44323,#44310,#36058,.T.);
#58640=EDGE_CURVE('',#44324,#44325,#36059,.T.);
#58641=EDGE_CURVE('',#44324,#44326,#36060,.T.);
#58642=EDGE_CURVE('',#44326,#44326,#36061,.T.);
#58643=EDGE_CURVE('',#44325,#44324,#36062,.T.);
#58644=EDGE_CURVE('',#44327,#44327,#36063,.T.);
#58645=EDGE_CURVE('',#44327,#44328,#36064,.T.);
#58646=EDGE_CURVE('',#44329,#44328,#36065,.T.);
#58647=EDGE_CURVE('',#44328,#44329,#36066,.T.);
#58648=EDGE_CURVE('',#44330,#44330,#5351,.T.);
#58649=EDGE_CURVE('',#44330,#44331,#24074,.T.);
#58650=EDGE_CURVE('',#44331,#44332,#5352,.T.);
#58651=EDGE_CURVE('',#44332,#44331,#5353,.T.);
#58652=EDGE_CURVE('',#44333,#44333,#36067,.T.);
#58653=EDGE_CURVE('',#44333,#44325,#24075,.T.);
#58654=EDGE_CURVE('',#44329,#44334,#24076,.T.);
#58655=EDGE_CURVE('',#44334,#44334,#36068,.T.);
#58656=EDGE_CURVE('',#44335,#44335,#36069,.T.);
#58657=EDGE_CURVE('',#44335,#44336,#36070,.T.);
#58658=EDGE_CURVE('',#44336,#44336,#36071,.T.);
#58659=EDGE_CURVE('',#44337,#44337,#36072,.T.);
#58660=EDGE_CURVE('',#44337,#44338,#36073,.T.);
#58661=EDGE_CURVE('',#44339,#44338,#36074,.T.);
#58662=EDGE_CURVE('',#44338,#44339,#36075,.T.);
#58663=EDGE_CURVE('',#44340,#44341,#36076,.T.);
#58664=EDGE_CURVE('',#44341,#44340,#36077,.T.);
#58665=EDGE_CURVE('',#44341,#44342,#36078,.T.);
#58666=EDGE_CURVE('',#44342,#44342,#36079,.T.);
#58667=EDGE_CURVE('',#44343,#44343,#36080,.T.);
#58668=EDGE_CURVE('',#44343,#44344,#36081,.T.);
#58669=EDGE_CURVE('',#44344,#44344,#36082,.T.);
#58670=EDGE_CURVE('',#44345,#44345,#36083,.T.);
#58671=EDGE_CURVE('',#44345,#44346,#36084,.T.);
#58672=EDGE_CURVE('',#44346,#44346,#36085,.T.);
#58673=EDGE_CURVE('',#44347,#44347,#36086,.T.);
#58674=EDGE_CURVE('',#44347,#44348,#24077,.T.);
#58675=EDGE_CURVE('',#44348,#44348,#36087,.T.);
#58676=EDGE_CURVE('',#44336,#44343,#24078,.T.);
#58677=EDGE_CURVE('',#44346,#44347,#24079,.T.);
#58678=EDGE_CURVE('',#44349,#44349,#36088,.T.);
#58679=EDGE_CURVE('',#44349,#44339,#24080,.T.);
#58680=EDGE_CURVE('',#44340,#44350,#24081,.T.);
#58681=EDGE_CURVE('',#44350,#44350,#36089,.T.);
#58682=EDGE_CURVE('',#44351,#44351,#36090,.T.);
#58683=EDGE_CURVE('',#44351,#44352,#24082,.T.);
#58684=EDGE_CURVE('',#44352,#44352,#36091,.T.);
#58685=EDGE_CURVE('',#44353,#44354,#24083,.T.);
#58686=EDGE_CURVE('',#44353,#44355,#4109,.T.);
#58687=EDGE_CURVE('',#44355,#44356,#2500,.T.);
#58688=EDGE_CURVE('',#44354,#44356,#4110,.T.);
#58689=EDGE_CURVE('',#44357,#44358,#24084,.T.);
#58690=EDGE_CURVE('',#44357,#44353,#4111,.T.);
#58691=EDGE_CURVE('',#44358,#44354,#4112,.T.);
#58692=EDGE_CURVE('',#44359,#44360,#24085,.T.);
#58693=EDGE_CURVE('',#44359,#44357,#4113,.T.);
#58694=EDGE_CURVE('',#44360,#44358,#4114,.T.);
#58695=EDGE_CURVE('',#44361,#44362,#24086,.T.);
#58696=EDGE_CURVE('',#44361,#44359,#4115,.T.);
#58697=EDGE_CURVE('',#44362,#44360,#4116,.T.);
#58698=EDGE_CURVE('',#44363,#44364,#24087,.T.);
#58699=EDGE_CURVE('',#44363,#44361,#4117,.T.);
#58700=EDGE_CURVE('',#44364,#44362,#4118,.T.);
#58701=EDGE_CURVE('',#44365,#44366,#24088,.T.);
#58702=EDGE_CURVE('',#44365,#44363,#4119,.T.);
#58703=EDGE_CURVE('',#44366,#44364,#4120,.T.);
#58704=EDGE_CURVE('',#44367,#44368,#24089,.T.);
#58705=EDGE_CURVE('',#44369,#44367,#5354,.F.);
#58706=EDGE_CURVE('',#44369,#44368,#36092,.T.);
#58707=EDGE_CURVE('',#44370,#44371,#24090,.T.);
#58708=EDGE_CURVE('',#44367,#44370,#5355,.F.);
#58709=EDGE_CURVE('',#44368,#44372,#36093,.T.);
#58710=EDGE_CURVE('',#44371,#44372,#5356,.F.);
#58711=EDGE_CURVE('',#44373,#44374,#24091,.T.);
#58712=EDGE_CURVE('',#44370,#44373,#5357,.F.);
#58713=EDGE_CURVE('',#44374,#44371,#5358,.F.);
#58714=EDGE_CURVE('',#44375,#44376,#24092,.T.);
#58715=EDGE_CURVE('',#44373,#44375,#5359,.F.);
#58716=EDGE_CURVE('',#44376,#44374,#5360,.F.);
#58717=EDGE_CURVE('',#44377,#44378,#24093,.T.);
#58718=EDGE_CURVE('',#44375,#44377,#5361,.F.);
#58719=EDGE_CURVE('',#44378,#44376,#5362,.F.);
#58720=EDGE_CURVE('',#44379,#44380,#24094,.T.);
#58721=EDGE_CURVE('',#44377,#44379,#5363,.F.);
#58722=EDGE_CURVE('',#44380,#44378,#5364,.F.);
#58723=EDGE_CURVE('',#44381,#44382,#24095,.T.);
#58724=EDGE_CURVE('',#44379,#44381,#5365,.F.);
#58725=EDGE_CURVE('',#44382,#44380,#5366,.F.);
#58726=EDGE_CURVE('',#44383,#44384,#24096,.T.);
#58727=EDGE_CURVE('',#44383,#44385,#36094,.T.);
#58728=EDGE_CURVE('',#44381,#44385,#5367,.F.);
#58729=EDGE_CURVE('',#44384,#44382,#5368,.F.);
#58730=EDGE_CURVE('',#44386,#44369,#36095,.T.);
#58731=EDGE_CURVE('',#44387,#44386,#36096,.T.);
#58732=EDGE_CURVE('',#44372,#44387,#36097,.T.);
#58733=EDGE_CURVE('',#44368,#44388,#24097,.T.);
#58734=EDGE_CURVE('',#44388,#44388,#36098,.T.);
#58735=EDGE_CURVE('',#44389,#44390,#36099,.T.);
#58736=EDGE_CURVE('',#44356,#44389,#36100,.T.);
#58737=EDGE_CURVE('',#44385,#44355,#36101,.T.);
#58738=EDGE_CURVE('',#44390,#44383,#36102,.T.);
#58739=EDGE_CURVE('',#44390,#44391,#24098,.T.);
#58740=EDGE_CURVE('',#44391,#44391,#36103,.T.);
#58741=EDGE_CURVE('',#44389,#44384,#5369,.F.);
#58742=EDGE_CURVE('',#44392,#44393,#36104,.T.);
#58743=EDGE_CURVE('',#44394,#44392,#36105,.T.);
#58744=EDGE_CURVE('',#44395,#44394,#36106,.T.);
#58745=EDGE_CURVE('',#44396,#44395,#36107,.T.);
#58746=EDGE_CURVE('',#44397,#44396,#36108,.T.);
#58747=EDGE_CURVE('',#44393,#44397,#36109,.T.);
#58748=EDGE_CURVE('',#44392,#44393,#4121,.T.);
#58749=EDGE_CURVE('',#44393,#44397,#4122,.T.);
#58750=EDGE_CURVE('',#44397,#44396,#4123,.T.);
#58751=EDGE_CURVE('',#44396,#44395,#4124,.T.);
#58752=EDGE_CURVE('',#44395,#44394,#4125,.T.);
#58753=EDGE_CURVE('',#44394,#44392,#4126,.T.);
#58754=EDGE_CURVE('',#44398,#44399,#24099,.T.);
#58755=EDGE_CURVE('',#44399,#44400,#24100,.T.);
#58756=EDGE_CURVE('',#44400,#44401,#24101,.T.);
#58757=EDGE_CURVE('',#44401,#44402,#24102,.T.);
#58758=EDGE_CURVE('',#44402,#44403,#24103,.T.);
#58759=EDGE_CURVE('',#44403,#44398,#24104,.T.);
#58760=EDGE_CURVE('',#44399,#44392,#24105,.T.);
#58761=EDGE_CURVE('',#44400,#44393,#24106,.T.);
#58762=EDGE_CURVE('',#44401,#44397,#24107,.T.);
#58763=EDGE_CURVE('',#44402,#44396,#24108,.T.);
#58764=EDGE_CURVE('',#44403,#44395,#24109,.T.);
#58765=EDGE_CURVE('',#44398,#44394,#24110,.T.);
#58766=EDGE_CURVE('',#44387,#44366,#4127,.T.);
#58767=EDGE_CURVE('',#44386,#44365,#4128,.T.);
#58768=EDGE_CURVE('',#44404,#44405,#24111,.T.);
#58769=EDGE_CURVE('',#44404,#44406,#4129,.T.);
#58770=EDGE_CURVE('',#44406,#44407,#36110,.T.);
#58771=EDGE_CURVE('',#44405,#44407,#4130,.T.);
#58772=EDGE_CURVE('',#44408,#44409,#24112,.T.);
#58773=EDGE_CURVE('',#44408,#44404,#4131,.T.);
#58774=EDGE_CURVE('',#44409,#44405,#4132,.T.);
#58775=EDGE_CURVE('',#44410,#44411,#24113,.T.);
#58776=EDGE_CURVE('',#44410,#44408,#4133,.T.);
#58777=EDGE_CURVE('',#44411,#44409,#4134,.T.);
#58778=EDGE_CURVE('',#44412,#44413,#24114,.T.);
#58779=EDGE_CURVE('',#44412,#44410,#4135,.T.);
#58780=EDGE_CURVE('',#44413,#44411,#4136,.T.);
#58781=EDGE_CURVE('',#44414,#44415,#24115,.T.);
#58782=EDGE_CURVE('',#44414,#44412,#4137,.T.);
#58783=EDGE_CURVE('',#44415,#44413,#4138,.T.);
#58784=EDGE_CURVE('',#44416,#44417,#24116,.T.);
#58785=EDGE_CURVE('',#44416,#44414,#4139,.T.);
#58786=EDGE_CURVE('',#44417,#44415,#4140,.T.);
#58787=EDGE_CURVE('',#44418,#44419,#24117,.T.);
#58788=EDGE_CURVE('',#44420,#44418,#5370,.F.);
#58789=EDGE_CURVE('',#44420,#44419,#36111,.T.);
#58790=EDGE_CURVE('',#44421,#44422,#24118,.T.);
#58791=EDGE_CURVE('',#44418,#44421,#5371,.F.);
#58792=EDGE_CURVE('',#44419,#44423,#36112,.T.);
#58793=EDGE_CURVE('',#44422,#44423,#5372,.F.);
#58794=EDGE_CURVE('',#44424,#44425,#24119,.T.);
#58795=EDGE_CURVE('',#44421,#44424,#5373,.F.);
#58796=EDGE_CURVE('',#44425,#44422,#5374,.F.);
#58797=EDGE_CURVE('',#44426,#44427,#24120,.T.);
#58798=EDGE_CURVE('',#44424,#44426,#5375,.F.);
#58799=EDGE_CURVE('',#44427,#44425,#5376,.F.);
#58800=EDGE_CURVE('',#44428,#44429,#24121,.T.);
#58801=EDGE_CURVE('',#44426,#44428,#5377,.F.);
#58802=EDGE_CURVE('',#44429,#44427,#5378,.F.);
#58803=EDGE_CURVE('',#44430,#44431,#24122,.T.);
#58804=EDGE_CURVE('',#44428,#44430,#5379,.F.);
#58805=EDGE_CURVE('',#44431,#44429,#5380,.F.);
#58806=EDGE_CURVE('',#44432,#44433,#24123,.T.);
#58807=EDGE_CURVE('',#44430,#44432,#5381,.F.);
#58808=EDGE_CURVE('',#44433,#44431,#5382,.F.);
#58809=EDGE_CURVE('',#44434,#44435,#24124,.T.);
#58810=EDGE_CURVE('',#44434,#44436,#36113,.T.);
#58811=EDGE_CURVE('',#44432,#44436,#5383,.F.);
#58812=EDGE_CURVE('',#44435,#44433,#5384,.F.);
#58813=EDGE_CURVE('',#44437,#44420,#36114,.T.);
#58814=EDGE_CURVE('',#44438,#44437,#36115,.T.);
#58815=EDGE_CURVE('',#44423,#44438,#36116,.T.);
#58816=EDGE_CURVE('',#44419,#44439,#24125,.T.);
#58817=EDGE_CURVE('',#44439,#44439,#36117,.T.);
#58818=EDGE_CURVE('',#44440,#44441,#36118,.T.);
#58819=EDGE_CURVE('',#44407,#44440,#36119,.T.);
#58820=EDGE_CURVE('',#44436,#44406,#36120,.T.);
#58821=EDGE_CURVE('',#44441,#44434,#36121,.T.);
#58822=EDGE_CURVE('',#44441,#44442,#24126,.T.);
#58823=EDGE_CURVE('',#44442,#44442,#36122,.T.);
#58824=EDGE_CURVE('',#44440,#44435,#5385,.F.);
#58825=EDGE_CURVE('',#44443,#44444,#36123,.T.);
#58826=EDGE_CURVE('',#44445,#44443,#36124,.T.);
#58827=EDGE_CURVE('',#44446,#44445,#36125,.T.);
#58828=EDGE_CURVE('',#44447,#44446,#36126,.T.);
#58829=EDGE_CURVE('',#44448,#44447,#36127,.T.);
#58830=EDGE_CURVE('',#44444,#44448,#36128,.T.);
#58831=EDGE_CURVE('',#44443,#44444,#4141,.T.);
#58832=EDGE_CURVE('',#44444,#44448,#4142,.T.);
#58833=EDGE_CURVE('',#44448,#44447,#4143,.T.);
#58834=EDGE_CURVE('',#44447,#44446,#4144,.T.);
#58835=EDGE_CURVE('',#44446,#44445,#4145,.T.);
#58836=EDGE_CURVE('',#44445,#44443,#4146,.T.);
#58837=EDGE_CURVE('',#44449,#44450,#24127,.T.);
#58838=EDGE_CURVE('',#44450,#44451,#24128,.T.);
#58839=EDGE_CURVE('',#44451,#44452,#24129,.T.);
#58840=EDGE_CURVE('',#44452,#44453,#24130,.T.);
#58841=EDGE_CURVE('',#44453,#44454,#24131,.T.);
#58842=EDGE_CURVE('',#44454,#44449,#24132,.T.);
#58843=EDGE_CURVE('',#44450,#44443,#24133,.T.);
#58844=EDGE_CURVE('',#44451,#44444,#24134,.T.);
#58845=EDGE_CURVE('',#44452,#44448,#24135,.T.);
#58846=EDGE_CURVE('',#44453,#44447,#24136,.T.);
#58847=EDGE_CURVE('',#44454,#44446,#24137,.T.);
#58848=EDGE_CURVE('',#44449,#44445,#24138,.T.);
#58849=EDGE_CURVE('',#44438,#44417,#4147,.T.);
#58850=EDGE_CURVE('',#44437,#44416,#4148,.T.);
#58851=EDGE_CURVE('',#44455,#44455,#36129,.T.);
#58852=EDGE_CURVE('',#44455,#44456,#24139,.T.);
#58853=EDGE_CURVE('',#44456,#44456,#36130,.T.);
#58854=EDGE_CURVE('',#44457,#44458,#36131,.T.);
#58855=EDGE_CURVE('',#44458,#44457,#36132,.T.);
#58856=EDGE_CURVE('',#44458,#44459,#24140,.T.);
#58857=EDGE_CURVE('',#44459,#44459,#36133,.T.);
#58858=EDGE_CURVE('',#44460,#44460,#36134,.T.);
#58859=EDGE_CURVE('',#44460,#44461,#24141,.T.);
#58860=EDGE_CURVE('',#44461,#44461,#36135,.T.);
#58861=EDGE_CURVE('',#44462,#44463,#36136,.T.);
#58862=EDGE_CURVE('',#44463,#44462,#36137,.T.);
#58863=EDGE_CURVE('',#44463,#44464,#24142,.T.);
#58864=EDGE_CURVE('',#44464,#44464,#36138,.T.);
#58865=EDGE_CURVE('',#44462,#44465,#24143,.T.);
#58866=EDGE_CURVE('',#44466,#44465,#5386,.T.);
#58867=EDGE_CURVE('',#44466,#44460,#24144,.T.);
#58868=EDGE_CURVE('',#44465,#44466,#5387,.T.);
#58869=EDGE_CURVE('',#44467,#44468,#5388,.T.);
#58870=EDGE_CURVE('',#44468,#44467,#5389,.T.);
#58871=EDGE_CURVE('',#44468,#44469,#24145,.T.);
#58872=EDGE_CURVE('',#44469,#44469,#5390,.T.);
#58873=EDGE_CURVE('',#44466,#44470,#24146,.T.);
#58874=EDGE_CURVE('',#44471,#44470,#5391,.T.);
#58875=EDGE_CURVE('',#44470,#44471,#5392,.T.);
#58876=EDGE_CURVE('',#44457,#44470,#24147,.T.);
#58877=EDGE_CURVE('',#44471,#44455,#24148,.T.);
#58878=EDGE_CURVE('',#44472,#44472,#36139,.T.);
#58879=EDGE_CURVE('',#44472,#44473,#24149,.T.);
#58880=EDGE_CURVE('',#44473,#44473,#36140,.T.);
#58881=EDGE_CURVE('',#44474,#44474,#36141,.T.);
#58882=EDGE_CURVE('',#44474,#44475,#24150,.T.);
#58883=EDGE_CURVE('',#44475,#44475,#36142,.T.);
#58884=EDGE_CURVE('',#44476,#44476,#36143,.T.);
#58885=EDGE_CURVE('',#44476,#44477,#36144,.T.);
#58886=EDGE_CURVE('',#44478,#44477,#36145,.T.);
#58887=EDGE_CURVE('',#44477,#44478,#36146,.T.);
#58888=EDGE_CURVE('',#44479,#44479,#36147,.T.);
#58889=EDGE_CURVE('',#44479,#44478,#24151,.T.);
#58890=EDGE_CURVE('',#44480,#44481,#36148,.T.);
#58891=EDGE_CURVE('',#44482,#44481,#24152,.T.);
#58892=EDGE_CURVE('',#44482,#44483,#36149,.T.);
#58893=EDGE_CURVE('',#44483,#44480,#24153,.T.);
#58894=EDGE_CURVE('',#44484,#44484,#36150,.T.);
#58895=EDGE_CURVE('',#44484,#44485,#24154,.T.);
#58896=EDGE_CURVE('',#44485,#44485,#36151,.T.);
#58897=EDGE_CURVE('',#44486,#44486,#36152,.T.);
#58898=EDGE_CURVE('',#44486,#44487,#24155,.T.);
#58899=EDGE_CURVE('',#44487,#44487,#36153,.T.);
#58900=EDGE_CURVE('',#44488,#44488,#36154,.T.);
#58901=EDGE_CURVE('',#44488,#44489,#24156,.T.);
#58902=EDGE_CURVE('',#44489,#44489,#36155,.T.);
#58903=EDGE_CURVE('',#44490,#44490,#36156,.T.);
#58904=EDGE_CURVE('',#44490,#44491,#24157,.T.);
#58905=EDGE_CURVE('',#44491,#44491,#36157,.T.);
#58906=EDGE_CURVE('',#44492,#44492,#36158,.T.);
#58907=EDGE_CURVE('',#44492,#44493,#24158,.T.);
#58908=EDGE_CURVE('',#44493,#44493,#36159,.T.);
#58909=EDGE_CURVE('',#44494,#44494,#36160,.T.);
#58910=EDGE_CURVE('',#44494,#44495,#24159,.T.);
#58911=EDGE_CURVE('',#44495,#44495,#36161,.T.);
#58912=EDGE_CURVE('',#44496,#44496,#36162,.T.);
#58913=EDGE_CURVE('',#44496,#44497,#24160,.T.);
#58914=EDGE_CURVE('',#44497,#44497,#36163,.T.);
#58915=EDGE_CURVE('',#44498,#44498,#36164,.T.);
#58916=EDGE_CURVE('',#44498,#44499,#24161,.T.);
#58917=EDGE_CURVE('',#44499,#44499,#36165,.T.);
#58918=EDGE_CURVE('',#44500,#44500,#36166,.T.);
#58919=EDGE_CURVE('',#44500,#44501,#24162,.T.);
#58920=EDGE_CURVE('',#44501,#44501,#36167,.T.);
#58921=EDGE_CURVE('',#44502,#44502,#36168,.T.);
#58922=EDGE_CURVE('',#44502,#44503,#24163,.T.);
#58923=EDGE_CURVE('',#44503,#44503,#36169,.T.);
#58924=EDGE_CURVE('',#44504,#44505,#24164,.T.);
#58925=EDGE_CURVE('',#44505,#44506,#36170,.T.);
#58926=EDGE_CURVE('',#44507,#44506,#24165,.T.);
#58927=EDGE_CURVE('',#44504,#44507,#36171,.T.);
#58928=EDGE_CURVE('',#44506,#44508,#24166,.T.);
#58929=EDGE_CURVE('',#44509,#44508,#24167,.T.);
#58930=EDGE_CURVE('',#44507,#44509,#24168,.T.);
#58931=EDGE_CURVE('',#44508,#44510,#36172,.T.);
#58932=EDGE_CURVE('',#44511,#44510,#24169,.T.);
#58933=EDGE_CURVE('',#44509,#44511,#36173,.T.);
#58934=EDGE_CURVE('',#44510,#44512,#24170,.T.);
#58935=EDGE_CURVE('',#44513,#44512,#24171,.T.);
#58936=EDGE_CURVE('',#44511,#44513,#24172,.T.);
#58937=EDGE_CURVE('',#44512,#44514,#36174,.T.);
#58938=EDGE_CURVE('',#44515,#44514,#24173,.T.);
#58939=EDGE_CURVE('',#44513,#44515,#36175,.T.);
#58940=EDGE_CURVE('',#44514,#44516,#24174,.T.);
#58941=EDGE_CURVE('',#44517,#44516,#24175,.T.);
#58942=EDGE_CURVE('',#44515,#44517,#24176,.T.);
#58943=EDGE_CURVE('',#44516,#44518,#36176,.T.);
#58944=EDGE_CURVE('',#44519,#44518,#24177,.T.);
#58945=EDGE_CURVE('',#44517,#44519,#36177,.T.);
#58946=EDGE_CURVE('',#44518,#44505,#24178,.T.);
#58947=EDGE_CURVE('',#44519,#44504,#24179,.T.);
#58948=EDGE_CURVE('',#44520,#44521,#24180,.T.);
#58949=EDGE_CURVE('',#44521,#44522,#36178,.T.);
#58950=EDGE_CURVE('',#44522,#44523,#24181,.T.);
#58951=EDGE_CURVE('',#44523,#44524,#36179,.T.);
#58952=EDGE_CURVE('',#44524,#44525,#24182,.T.);
#58953=EDGE_CURVE('',#44525,#44526,#36180,.T.);
#58954=EDGE_CURVE('',#44526,#44527,#24183,.T.);
#58955=EDGE_CURVE('',#44527,#44520,#36181,.T.);
#58956=EDGE_CURVE('',#44528,#44529,#36182,.T.);
#58957=EDGE_CURVE('',#44530,#44528,#24184,.T.);
#58958=EDGE_CURVE('',#44531,#44530,#36183,.T.);
#58959=EDGE_CURVE('',#44532,#44531,#24185,.T.);
#58960=EDGE_CURVE('',#44533,#44532,#36184,.T.);
#58961=EDGE_CURVE('',#44534,#44533,#24186,.T.);
#58962=EDGE_CURVE('',#44535,#44534,#36185,.T.);
#58963=EDGE_CURVE('',#44529,#44535,#24187,.T.);
#58964=EDGE_CURVE('',#44536,#44529,#24188,.T.);
#58965=EDGE_CURVE('',#44537,#44536,#36186,.T.);
#58966=EDGE_CURVE('',#44537,#44528,#24189,.T.);
#58967=EDGE_CURVE('',#44538,#44535,#24190,.T.);
#58968=EDGE_CURVE('',#44536,#44538,#24191,.T.);
#58969=EDGE_CURVE('',#44539,#44534,#24192,.T.);
#58970=EDGE_CURVE('',#44538,#44539,#36187,.T.);
#58971=EDGE_CURVE('',#44540,#44533,#24193,.T.);
#58972=EDGE_CURVE('',#44539,#44540,#24194,.T.);
#58973=EDGE_CURVE('',#44541,#44532,#24195,.T.);
#58974=EDGE_CURVE('',#44540,#44541,#36188,.T.);
#58975=EDGE_CURVE('',#44542,#44531,#24196,.T.);
#58976=EDGE_CURVE('',#44541,#44542,#24197,.T.);
#58977=EDGE_CURVE('',#44543,#44530,#24198,.T.);
#58978=EDGE_CURVE('',#44542,#44543,#36189,.T.);
#58979=EDGE_CURVE('',#44543,#44537,#24199,.T.);
#58980=EDGE_CURVE('',#44526,#44512,#36190,.T.);
#58981=EDGE_CURVE('',#44514,#44525,#36191,.T.);
#58982=EDGE_CURVE('',#44516,#44524,#36192,.T.);
#58983=EDGE_CURVE('',#44527,#44510,#36193,.T.);
#58984=EDGE_CURVE('',#44518,#44523,#36194,.T.);
#58985=EDGE_CURVE('',#44520,#44508,#36195,.T.);
#58986=EDGE_CURVE('',#44505,#44522,#36196,.T.);
#58987=EDGE_CURVE('',#44521,#44506,#36197,.T.);
#58988=EDGE_CURVE('',#44544,#44545,#24200,.T.);
#58989=EDGE_CURVE('',#44545,#44546,#36198,.T.);
#58990=EDGE_CURVE('',#44547,#44546,#24201,.T.);
#58991=EDGE_CURVE('',#44547,#44544,#36199,.T.);
#58992=EDGE_CURVE('',#44545,#44548,#24202,.T.);
#58993=EDGE_CURVE('',#44548,#44549,#36200,.T.);
#58994=EDGE_CURVE('',#44549,#44481,#24203,.T.);
#58995=EDGE_CURVE('',#44550,#44480,#24204,.T.);
#58996=EDGE_CURVE('',#44551,#44550,#36201,.T.);
#58997=EDGE_CURVE('',#44546,#44551,#24205,.T.);
#58998=EDGE_CURVE('',#44552,#44550,#24206,.T.);
#58999=EDGE_CURVE('',#44553,#44552,#36202,.T.);
#59000=EDGE_CURVE('',#44553,#44551,#24207,.T.);
#59001=EDGE_CURVE('',#44547,#44553,#24208,.T.);
#59002=EDGE_CURVE('',#44552,#44483,#24209,.T.);
#59003=EDGE_CURVE('',#44554,#44482,#24210,.T.);
#59004=EDGE_CURVE('',#44555,#44554,#36203,.T.);
#59005=EDGE_CURVE('',#44544,#44555,#24211,.T.);
#59006=EDGE_CURVE('',#44555,#44548,#24212,.T.);
#59007=EDGE_CURVE('',#44554,#44549,#24213,.T.);
#60937=ORIENTED_EDGE('',*,*,#45747,.F.);
#60938=ORIENTED_EDGE('',*,*,#45748,.T.);
#60939=ORIENTED_EDGE('',*,*,#45749,.T.);
#60940=ORIENTED_EDGE('',*,*,#45750,.T.);
#60941=ORIENTED_EDGE('',*,*,#45748,.F.);
#60942=ORIENTED_EDGE('',*,*,#45751,.F.);
#60943=ORIENTED_EDGE('',*,*,#45752,.F.);
#60944=ORIENTED_EDGE('',*,*,#45753,.F.);
#60945=ORIENTED_EDGE('',*,*,#45754,.F.);
#60946=ORIENTED_EDGE('',*,*,#45755,.F.);
#60947=ORIENTED_EDGE('',*,*,#45756,.F.);
#60948=ORIENTED_EDGE('',*,*,#45753,.T.);
#60949=ORIENTED_EDGE('',*,*,#45757,.F.);
#60950=ORIENTED_EDGE('',*,*,#45758,.F.);
#60951=ORIENTED_EDGE('',*,*,#45759,.T.);
#60952=ORIENTED_EDGE('',*,*,#45760,.T.);
#60953=ORIENTED_EDGE('',*,*,#45759,.F.);
#60954=ORIENTED_EDGE('',*,*,#45761,.F.);
#60955=ORIENTED_EDGE('',*,*,#45762,.F.);
#60956=ORIENTED_EDGE('',*,*,#45763,.T.);
#60957=ORIENTED_EDGE('',*,*,#45764,.F.);
#60958=ORIENTED_EDGE('',*,*,#45765,.F.);
#60959=ORIENTED_EDGE('',*,*,#45766,.T.);
#60960=ORIENTED_EDGE('',*,*,#45767,.T.);
#60961=ORIENTED_EDGE('',*,*,#45768,.T.);
#60962=ORIENTED_EDGE('',*,*,#45761,.T.);
#60963=ORIENTED_EDGE('',*,*,#45769,.T.);
#60964=ORIENTED_EDGE('',*,*,#45749,.F.);
#60965=ORIENTED_EDGE('',*,*,#45750,.F.);
#60966=ORIENTED_EDGE('',*,*,#45769,.F.);
#60967=ORIENTED_EDGE('',*,*,#45765,.T.);
#60968=ORIENTED_EDGE('',*,*,#45770,.T.);
#60969=ORIENTED_EDGE('',*,*,#45771,.T.);
#60970=ORIENTED_EDGE('',*,*,#45772,.F.);
#60971=ORIENTED_EDGE('',*,*,#45747,.T.);
#60972=ORIENTED_EDGE('',*,*,#45773,.F.);
#60973=ORIENTED_EDGE('',*,*,#45774,.F.);
#60974=ORIENTED_EDGE('',*,*,#45775,.T.);
#60975=ORIENTED_EDGE('',*,*,#45772,.T.);
#60976=ORIENTED_EDGE('',*,*,#45775,.F.);
#60977=ORIENTED_EDGE('',*,*,#45773,.T.);
#60978=ORIENTED_EDGE('',*,*,#45774,.T.);
#60979=ORIENTED_EDGE('',*,*,#45776,.T.);
#60980=ORIENTED_EDGE('',*,*,#45777,.F.);
#60981=ORIENTED_EDGE('',*,*,#45778,.F.);
#60982=ORIENTED_EDGE('',*,*,#45776,.F.);
#60983=ORIENTED_EDGE('',*,*,#45779,.F.);
#60984=ORIENTED_EDGE('',*,*,#45780,.T.);
#60985=ORIENTED_EDGE('',*,*,#45777,.T.);
#60986=ORIENTED_EDGE('',*,*,#45778,.T.);
#60987=ORIENTED_EDGE('',*,*,#45780,.F.);
#60988=ORIENTED_EDGE('',*,*,#45781,.F.);
#60989=ORIENTED_EDGE('',*,*,#45782,.T.);
#60990=ORIENTED_EDGE('',*,*,#45783,.T.);
#60991=ORIENTED_EDGE('',*,*,#45782,.F.);
#60992=ORIENTED_EDGE('',*,*,#45779,.T.);
#60993=ORIENTED_EDGE('',*,*,#45783,.F.);
#60994=ORIENTED_EDGE('',*,*,#45781,.T.);
#60995=ORIENTED_EDGE('',*,*,#45784,.F.);
#60996=ORIENTED_EDGE('',*,*,#45751,.T.);
#60997=ORIENTED_EDGE('',*,*,#45785,.F.);
#60998=ORIENTED_EDGE('',*,*,#45766,.F.);
#60999=ORIENTED_EDGE('',*,*,#45786,.F.);
#61000=ORIENTED_EDGE('',*,*,#45787,.T.);
#61001=ORIENTED_EDGE('',*,*,#45788,.F.);
#61002=ORIENTED_EDGE('',*,*,#45771,.F.);
#61003=ORIENTED_EDGE('',*,*,#45789,.F.);
#61004=ORIENTED_EDGE('',*,*,#45790,.T.);
#61005=ORIENTED_EDGE('',*,*,#45791,.F.);
#61006=ORIENTED_EDGE('',*,*,#45770,.F.);
#61007=ORIENTED_EDGE('',*,*,#45792,.F.);
#61008=ORIENTED_EDGE('',*,*,#45793,.T.);
#61009=ORIENTED_EDGE('',*,*,#45794,.F.);
#61010=ORIENTED_EDGE('',*,*,#45768,.F.);
#61011=ORIENTED_EDGE('',*,*,#45795,.F.);
#61012=ORIENTED_EDGE('',*,*,#45796,.T.);
#61013=ORIENTED_EDGE('',*,*,#45797,.F.);
#61014=ORIENTED_EDGE('',*,*,#45767,.F.);
#61015=ORIENTED_EDGE('',*,*,#45760,.F.);
#61016=ORIENTED_EDGE('',*,*,#45755,.T.);
#61017=ORIENTED_EDGE('',*,*,#45798,.T.);
#61018=ORIENTED_EDGE('',*,*,#45799,.T.);
#61019=ORIENTED_EDGE('',*,*,#45800,.T.);
#61020=ORIENTED_EDGE('',*,*,#45801,.T.);
#61021=ORIENTED_EDGE('',*,*,#45802,.T.);
#61022=ORIENTED_EDGE('',*,*,#45758,.T.);
#61023=ORIENTED_EDGE('',*,*,#45803,.F.);
#61024=ORIENTED_EDGE('',*,*,#45804,.T.);
#61025=ORIENTED_EDGE('',*,*,#45805,.F.);
#61026=ORIENTED_EDGE('',*,*,#45802,.F.);
#61027=ORIENTED_EDGE('',*,*,#45806,.F.);
#61028=ORIENTED_EDGE('',*,*,#45807,.T.);
#61029=ORIENTED_EDGE('',*,*,#45808,.F.);
#61030=ORIENTED_EDGE('',*,*,#45801,.F.);
#61031=ORIENTED_EDGE('',*,*,#45809,.F.);
#61032=ORIENTED_EDGE('',*,*,#45810,.T.);
#61033=ORIENTED_EDGE('',*,*,#45811,.F.);
#61034=ORIENTED_EDGE('',*,*,#45800,.F.);
#61035=ORIENTED_EDGE('',*,*,#45812,.F.);
#61036=ORIENTED_EDGE('',*,*,#45813,.T.);
#61037=ORIENTED_EDGE('',*,*,#45814,.F.);
#61038=ORIENTED_EDGE('',*,*,#45799,.F.);
#61039=ORIENTED_EDGE('',*,*,#45815,.F.);
#61040=ORIENTED_EDGE('',*,*,#45816,.T.);
#61041=ORIENTED_EDGE('',*,*,#45817,.F.);
#61042=ORIENTED_EDGE('',*,*,#45798,.F.);
#61043=ORIENTED_EDGE('',*,*,#45788,.T.);
#61044=ORIENTED_EDGE('',*,*,#45818,.T.);
#61045=ORIENTED_EDGE('',*,*,#45815,.T.);
#61046=ORIENTED_EDGE('',*,*,#45757,.T.);
#61047=ORIENTED_EDGE('',*,*,#45752,.T.);
#61048=ORIENTED_EDGE('',*,*,#45784,.T.);
#61049=ORIENTED_EDGE('',*,*,#45817,.T.);
#61050=ORIENTED_EDGE('',*,*,#45819,.T.);
#61051=ORIENTED_EDGE('',*,*,#45786,.T.);
#61052=ORIENTED_EDGE('',*,*,#45791,.T.);
#61053=ORIENTED_EDGE('',*,*,#45820,.T.);
#61054=ORIENTED_EDGE('',*,*,#45812,.T.);
#61055=ORIENTED_EDGE('',*,*,#45814,.T.);
#61056=ORIENTED_EDGE('',*,*,#45821,.T.);
#61057=ORIENTED_EDGE('',*,*,#45789,.T.);
#61058=ORIENTED_EDGE('',*,*,#45764,.T.);
#61059=ORIENTED_EDGE('',*,*,#45822,.T.);
#61060=ORIENTED_EDGE('',*,*,#45809,.T.);
#61061=ORIENTED_EDGE('',*,*,#45794,.T.);
#61062=ORIENTED_EDGE('',*,*,#45823,.T.);
#61063=ORIENTED_EDGE('',*,*,#45806,.T.);
#61064=ORIENTED_EDGE('',*,*,#45811,.T.);
#61065=ORIENTED_EDGE('',*,*,#45824,.T.);
#61066=ORIENTED_EDGE('',*,*,#45762,.T.);
#61067=ORIENTED_EDGE('',*,*,#45797,.T.);
#61068=ORIENTED_EDGE('',*,*,#45825,.T.);
#61069=ORIENTED_EDGE('',*,*,#45803,.T.);
#61070=ORIENTED_EDGE('',*,*,#45808,.T.);
#61071=ORIENTED_EDGE('',*,*,#45826,.T.);
#61072=ORIENTED_EDGE('',*,*,#45792,.T.);
#61073=ORIENTED_EDGE('',*,*,#45785,.T.);
#61074=ORIENTED_EDGE('',*,*,#45754,.T.);
#61075=ORIENTED_EDGE('',*,*,#45756,.T.);
#61076=ORIENTED_EDGE('',*,*,#45805,.T.);
#61077=ORIENTED_EDGE('',*,*,#45827,.T.);
#61078=ORIENTED_EDGE('',*,*,#45795,.T.);
#61079=ORIENTED_EDGE('',*,*,#45787,.F.);
#61080=ORIENTED_EDGE('',*,*,#45819,.F.);
#61081=ORIENTED_EDGE('',*,*,#45816,.F.);
#61082=ORIENTED_EDGE('',*,*,#45818,.F.);
#61083=ORIENTED_EDGE('',*,*,#45796,.F.);
#61084=ORIENTED_EDGE('',*,*,#45827,.F.);
#61085=ORIENTED_EDGE('',*,*,#45804,.F.);
#61086=ORIENTED_EDGE('',*,*,#45825,.F.);
#61087=ORIENTED_EDGE('',*,*,#45793,.F.);
#61088=ORIENTED_EDGE('',*,*,#45826,.F.);
#61089=ORIENTED_EDGE('',*,*,#45807,.F.);
#61090=ORIENTED_EDGE('',*,*,#45823,.F.);
#61091=ORIENTED_EDGE('',*,*,#45790,.F.);
#61092=ORIENTED_EDGE('',*,*,#45821,.F.);
#61093=ORIENTED_EDGE('',*,*,#45813,.F.);
#61094=ORIENTED_EDGE('',*,*,#45820,.F.);
#61095=ORIENTED_EDGE('',*,*,#45763,.F.);
#61096=ORIENTED_EDGE('',*,*,#45824,.F.);
#61097=ORIENTED_EDGE('',*,*,#45810,.F.);
#61098=ORIENTED_EDGE('',*,*,#45822,.F.);
#61099=ORIENTED_EDGE('',*,*,#45828,.T.);
#61100=ORIENTED_EDGE('',*,*,#45829,.T.);
#61101=ORIENTED_EDGE('',*,*,#45830,.F.);
#61102=ORIENTED_EDGE('',*,*,#45829,.F.);
#61103=ORIENTED_EDGE('',*,*,#45831,.T.);
#61104=ORIENTED_EDGE('',*,*,#45832,.T.);
#61105=ORIENTED_EDGE('',*,*,#45833,.F.);
#61106=ORIENTED_EDGE('',*,*,#45832,.F.);
#61107=ORIENTED_EDGE('',*,*,#45831,.F.);
#61108=ORIENTED_EDGE('',*,*,#45830,.T.);
#61109=ORIENTED_EDGE('',*,*,#45833,.T.);
#61110=ORIENTED_EDGE('',*,*,#45828,.F.);
#61111=ORIENTED_EDGE('',*,*,#45834,.T.);
#61112=ORIENTED_EDGE('',*,*,#45835,.T.);
#61113=ORIENTED_EDGE('',*,*,#45836,.F.);
#61114=ORIENTED_EDGE('',*,*,#45835,.F.);
#61115=ORIENTED_EDGE('',*,*,#45837,.T.);
#61116=ORIENTED_EDGE('',*,*,#45838,.T.);
#61117=ORIENTED_EDGE('',*,*,#45839,.F.);
#61118=ORIENTED_EDGE('',*,*,#45838,.F.);
#61119=ORIENTED_EDGE('',*,*,#45837,.F.);
#61120=ORIENTED_EDGE('',*,*,#45836,.T.);
#61121=ORIENTED_EDGE('',*,*,#45839,.T.);
#61122=ORIENTED_EDGE('',*,*,#45834,.F.);
#61123=ORIENTED_EDGE('',*,*,#45840,.T.);
#61124=ORIENTED_EDGE('',*,*,#45841,.T.);
#61125=ORIENTED_EDGE('',*,*,#45842,.F.);
#61126=ORIENTED_EDGE('',*,*,#45841,.F.);
#61127=ORIENTED_EDGE('',*,*,#45843,.T.);
#61128=ORIENTED_EDGE('',*,*,#45844,.T.);
#61129=ORIENTED_EDGE('',*,*,#45845,.F.);
#61130=ORIENTED_EDGE('',*,*,#45844,.F.);
#61131=ORIENTED_EDGE('',*,*,#45843,.F.);
#61132=ORIENTED_EDGE('',*,*,#45842,.T.);
#61133=ORIENTED_EDGE('',*,*,#45845,.T.);
#61134=ORIENTED_EDGE('',*,*,#45840,.F.);
#61135=ORIENTED_EDGE('',*,*,#45846,.T.);
#61136=ORIENTED_EDGE('',*,*,#45847,.T.);
#61137=ORIENTED_EDGE('',*,*,#45848,.F.);
#61138=ORIENTED_EDGE('',*,*,#45847,.F.);
#61139=ORIENTED_EDGE('',*,*,#45849,.T.);
#61140=ORIENTED_EDGE('',*,*,#45850,.T.);
#61141=ORIENTED_EDGE('',*,*,#45851,.F.);
#61142=ORIENTED_EDGE('',*,*,#45850,.F.);
#61143=ORIENTED_EDGE('',*,*,#45849,.F.);
#61144=ORIENTED_EDGE('',*,*,#45848,.T.);
#61145=ORIENTED_EDGE('',*,*,#45851,.T.);
#61146=ORIENTED_EDGE('',*,*,#45846,.F.);
#61147=ORIENTED_EDGE('',*,*,#45852,.F.);
#61148=ORIENTED_EDGE('',*,*,#45853,.F.);
#61149=ORIENTED_EDGE('',*,*,#45854,.T.);
#61150=ORIENTED_EDGE('',*,*,#45855,.F.);
#61151=ORIENTED_EDGE('',*,*,#45854,.F.);
#61152=ORIENTED_EDGE('',*,*,#45856,.F.);
#61153=ORIENTED_EDGE('',*,*,#45857,.T.);
#61154=ORIENTED_EDGE('',*,*,#45858,.F.);
#61155=ORIENTED_EDGE('',*,*,#45859,.F.);
#61156=ORIENTED_EDGE('',*,*,#45857,.F.);
#61157=ORIENTED_EDGE('',*,*,#45860,.T.);
#61158=ORIENTED_EDGE('',*,*,#45861,.T.);
#61159=ORIENTED_EDGE('',*,*,#45858,.T.);
#61160=ORIENTED_EDGE('',*,*,#45859,.T.);
#61161=ORIENTED_EDGE('',*,*,#45861,.F.);
#61162=ORIENTED_EDGE('',*,*,#45852,.T.);
#61163=ORIENTED_EDGE('',*,*,#45853,.T.);
#61164=ORIENTED_EDGE('',*,*,#45862,.T.);
#61165=ORIENTED_EDGE('',*,*,#45863,.T.);
#61166=ORIENTED_EDGE('',*,*,#45862,.F.);
#61167=ORIENTED_EDGE('',*,*,#45860,.F.);
#61168=ORIENTED_EDGE('',*,*,#45863,.F.);
#61169=ORIENTED_EDGE('',*,*,#45856,.T.);
#61170=ORIENTED_EDGE('',*,*,#45855,.T.);
#61171=ORIENTED_EDGE('',*,*,#45864,.F.);
#61172=ORIENTED_EDGE('',*,*,#45865,.T.);
#61173=ORIENTED_EDGE('',*,*,#45866,.F.);
#61174=ORIENTED_EDGE('',*,*,#45867,.F.);
#61175=ORIENTED_EDGE('',*,*,#45865,.F.);
#61176=ORIENTED_EDGE('',*,*,#45868,.F.);
#61177=ORIENTED_EDGE('',*,*,#45869,.F.);
#61178=ORIENTED_EDGE('',*,*,#45870,.T.);
#61179=ORIENTED_EDGE('',*,*,#45871,.F.);
#61180=ORIENTED_EDGE('',*,*,#45870,.F.);
#61181=ORIENTED_EDGE('',*,*,#45872,.T.);
#61182=ORIENTED_EDGE('',*,*,#45873,.T.);
#61183=ORIENTED_EDGE('',*,*,#45866,.T.);
#61184=ORIENTED_EDGE('',*,*,#45867,.T.);
#61185=ORIENTED_EDGE('',*,*,#45873,.F.);
#61186=ORIENTED_EDGE('',*,*,#45868,.T.);
#61187=ORIENTED_EDGE('',*,*,#45869,.T.);
#61188=ORIENTED_EDGE('',*,*,#45874,.T.);
#61189=ORIENTED_EDGE('',*,*,#45875,.F.);
#61190=ORIENTED_EDGE('',*,*,#45874,.F.);
#61191=ORIENTED_EDGE('',*,*,#45872,.F.);
#61192=ORIENTED_EDGE('',*,*,#45875,.T.);
#61193=ORIENTED_EDGE('',*,*,#45864,.T.);
#61194=ORIENTED_EDGE('',*,*,#45871,.T.);
#61195=ORIENTED_EDGE('',*,*,#45876,.T.);
#61196=ORIENTED_EDGE('',*,*,#45877,.T.);
#61197=ORIENTED_EDGE('',*,*,#45878,.F.);
#61198=ORIENTED_EDGE('',*,*,#45877,.F.);
#61199=ORIENTED_EDGE('',*,*,#45879,.T.);
#61200=ORIENTED_EDGE('',*,*,#45880,.T.);
#61201=ORIENTED_EDGE('',*,*,#45881,.F.);
#61202=ORIENTED_EDGE('',*,*,#45880,.F.);
#61203=ORIENTED_EDGE('',*,*,#45879,.F.);
#61204=ORIENTED_EDGE('',*,*,#45878,.T.);
#61205=ORIENTED_EDGE('',*,*,#45881,.T.);
#61206=ORIENTED_EDGE('',*,*,#45876,.F.);
#61207=ORIENTED_EDGE('',*,*,#45882,.F.);
#61208=ORIENTED_EDGE('',*,*,#45883,.F.);
#61209=ORIENTED_EDGE('',*,*,#45884,.F.);
#61210=ORIENTED_EDGE('',*,*,#45885,.T.);
#61211=ORIENTED_EDGE('',*,*,#45886,.F.);
#61212=ORIENTED_EDGE('',*,*,#45887,.F.);
#61213=ORIENTED_EDGE('',*,*,#45888,.F.);
#61214=ORIENTED_EDGE('',*,*,#45889,.T.);
#61215=ORIENTED_EDGE('',*,*,#45890,.F.);
#61216=ORIENTED_EDGE('',*,*,#45891,.F.);
#61217=ORIENTED_EDGE('',*,*,#45892,.F.);
#61218=ORIENTED_EDGE('',*,*,#45893,.T.);
#61219=ORIENTED_EDGE('',*,*,#45894,.F.);
#61220=ORIENTED_EDGE('',*,*,#45895,.F.);
#61221=ORIENTED_EDGE('',*,*,#45896,.F.);
#61222=ORIENTED_EDGE('',*,*,#45897,.T.);
#61223=ORIENTED_EDGE('',*,*,#45898,.F.);
#61224=ORIENTED_EDGE('',*,*,#45899,.F.);
#61225=ORIENTED_EDGE('',*,*,#45900,.T.);
#61226=ORIENTED_EDGE('',*,*,#45901,.F.);
#61227=ORIENTED_EDGE('',*,*,#45902,.F.);
#61228=ORIENTED_EDGE('',*,*,#45900,.F.);
#61229=ORIENTED_EDGE('',*,*,#45903,.F.);
#61230=ORIENTED_EDGE('',*,*,#45904,.T.);
#61231=ORIENTED_EDGE('',*,*,#45905,.F.);
#61232=ORIENTED_EDGE('',*,*,#45904,.F.);
#61233=ORIENTED_EDGE('',*,*,#45906,.F.);
#61234=ORIENTED_EDGE('',*,*,#45907,.T.);
#61235=ORIENTED_EDGE('',*,*,#45908,.F.);
#61236=ORIENTED_EDGE('',*,*,#45909,.F.);
#61237=ORIENTED_EDGE('',*,*,#45907,.F.);
#61238=ORIENTED_EDGE('',*,*,#45910,.F.);
#61239=ORIENTED_EDGE('',*,*,#45911,.T.);
#61240=ORIENTED_EDGE('',*,*,#45912,.F.);
#61241=ORIENTED_EDGE('',*,*,#45911,.F.);
#61242=ORIENTED_EDGE('',*,*,#45913,.F.);
#61243=ORIENTED_EDGE('',*,*,#45914,.T.);
#61244=ORIENTED_EDGE('',*,*,#45915,.T.);
#61245=ORIENTED_EDGE('',*,*,#45914,.F.);
#61246=ORIENTED_EDGE('',*,*,#45915,.F.);
#61247=ORIENTED_EDGE('',*,*,#45916,.T.);
#61248=ORIENTED_EDGE('',*,*,#45910,.T.);
#61249=ORIENTED_EDGE('',*,*,#45916,.F.);
#61250=ORIENTED_EDGE('',*,*,#45917,.T.);
#61251=ORIENTED_EDGE('',*,*,#45918,.T.);
#61252=ORIENTED_EDGE('',*,*,#45919,.T.);
#61253=ORIENTED_EDGE('',*,*,#45920,.T.);
#61254=ORIENTED_EDGE('',*,*,#45921,.T.);
#61255=ORIENTED_EDGE('',*,*,#45922,.T.);
#61256=ORIENTED_EDGE('',*,*,#45923,.T.);
#61257=ORIENTED_EDGE('',*,*,#45924,.T.);
#61258=ORIENTED_EDGE('',*,*,#45925,.T.);
#61259=ORIENTED_EDGE('',*,*,#45926,.T.);
#61260=ORIENTED_EDGE('',*,*,#45927,.T.);
#61261=ORIENTED_EDGE('',*,*,#45928,.T.);
#61262=ORIENTED_EDGE('',*,*,#45929,.T.);
#61263=ORIENTED_EDGE('',*,*,#45930,.T.);
#61264=ORIENTED_EDGE('',*,*,#45931,.T.);
#61265=ORIENTED_EDGE('',*,*,#45932,.T.);
#61266=ORIENTED_EDGE('',*,*,#45933,.T.);
#61267=ORIENTED_EDGE('',*,*,#45934,.T.);
#61268=ORIENTED_EDGE('',*,*,#45935,.T.);
#61269=ORIENTED_EDGE('',*,*,#45936,.T.);
#61270=ORIENTED_EDGE('',*,*,#45937,.T.);
#61271=ORIENTED_EDGE('',*,*,#45938,.T.);
#61272=ORIENTED_EDGE('',*,*,#45939,.T.);
#61273=ORIENTED_EDGE('',*,*,#45940,.T.);
#61274=ORIENTED_EDGE('',*,*,#45941,.T.);
#61275=ORIENTED_EDGE('',*,*,#45942,.T.);
#61276=ORIENTED_EDGE('',*,*,#45943,.T.);
#61277=ORIENTED_EDGE('',*,*,#45944,.T.);
#61278=ORIENTED_EDGE('',*,*,#45945,.T.);
#61279=ORIENTED_EDGE('',*,*,#45946,.T.);
#61280=ORIENTED_EDGE('',*,*,#45947,.T.);
#61281=ORIENTED_EDGE('',*,*,#45948,.T.);
#61282=ORIENTED_EDGE('',*,*,#45949,.T.);
#61283=ORIENTED_EDGE('',*,*,#45950,.T.);
#61284=ORIENTED_EDGE('',*,*,#45951,.T.);
#61285=ORIENTED_EDGE('',*,*,#45952,.T.);
#61286=ORIENTED_EDGE('',*,*,#45953,.T.);
#61287=ORIENTED_EDGE('',*,*,#45954,.T.);
#61288=ORIENTED_EDGE('',*,*,#45955,.T.);
#61289=ORIENTED_EDGE('',*,*,#45956,.T.);
#61290=ORIENTED_EDGE('',*,*,#45957,.T.);
#61291=ORIENTED_EDGE('',*,*,#45958,.T.);
#61292=ORIENTED_EDGE('',*,*,#45959,.T.);
#61293=ORIENTED_EDGE('',*,*,#45960,.T.);
#61294=ORIENTED_EDGE('',*,*,#45961,.T.);
#61295=ORIENTED_EDGE('',*,*,#45962,.T.);
#61296=ORIENTED_EDGE('',*,*,#45963,.T.);
#61297=ORIENTED_EDGE('',*,*,#45964,.T.);
#61298=ORIENTED_EDGE('',*,*,#45965,.T.);
#61299=ORIENTED_EDGE('',*,*,#45966,.T.);
#61300=ORIENTED_EDGE('',*,*,#45967,.T.);
#61301=ORIENTED_EDGE('',*,*,#45968,.T.);
#61302=ORIENTED_EDGE('',*,*,#45969,.T.);
#61303=ORIENTED_EDGE('',*,*,#45970,.T.);
#61304=ORIENTED_EDGE('',*,*,#45971,.T.);
#61305=ORIENTED_EDGE('',*,*,#45972,.T.);
#61306=ORIENTED_EDGE('',*,*,#45973,.T.);
#61307=ORIENTED_EDGE('',*,*,#45974,.T.);
#61308=ORIENTED_EDGE('',*,*,#45975,.T.);
#61309=ORIENTED_EDGE('',*,*,#45976,.T.);
#61310=ORIENTED_EDGE('',*,*,#45977,.T.);
#61311=ORIENTED_EDGE('',*,*,#45978,.T.);
#61312=ORIENTED_EDGE('',*,*,#45979,.T.);
#61313=ORIENTED_EDGE('',*,*,#45980,.T.);
#61314=ORIENTED_EDGE('',*,*,#45981,.T.);
#61315=ORIENTED_EDGE('',*,*,#45982,.T.);
#61316=ORIENTED_EDGE('',*,*,#45983,.T.);
#61317=ORIENTED_EDGE('',*,*,#45984,.T.);
#61318=ORIENTED_EDGE('',*,*,#45985,.T.);
#61319=ORIENTED_EDGE('',*,*,#45986,.T.);
#61320=ORIENTED_EDGE('',*,*,#45987,.T.);
#61321=ORIENTED_EDGE('',*,*,#45988,.T.);
#61322=ORIENTED_EDGE('',*,*,#45989,.T.);
#61323=ORIENTED_EDGE('',*,*,#45990,.T.);
#61324=ORIENTED_EDGE('',*,*,#45991,.T.);
#61325=ORIENTED_EDGE('',*,*,#45992,.T.);
#61326=ORIENTED_EDGE('',*,*,#45993,.T.);
#61327=ORIENTED_EDGE('',*,*,#45994,.T.);
#61328=ORIENTED_EDGE('',*,*,#45995,.T.);
#61329=ORIENTED_EDGE('',*,*,#45996,.T.);
#61330=ORIENTED_EDGE('',*,*,#45997,.T.);
#61331=ORIENTED_EDGE('',*,*,#45998,.T.);
#61332=ORIENTED_EDGE('',*,*,#45999,.T.);
#61333=ORIENTED_EDGE('',*,*,#46000,.T.);
#61334=ORIENTED_EDGE('',*,*,#46001,.T.);
#61335=ORIENTED_EDGE('',*,*,#46002,.T.);
#61336=ORIENTED_EDGE('',*,*,#46003,.T.);
#61337=ORIENTED_EDGE('',*,*,#46004,.T.);
#61338=ORIENTED_EDGE('',*,*,#46005,.T.);
#61339=ORIENTED_EDGE('',*,*,#46006,.T.);
#61340=ORIENTED_EDGE('',*,*,#46007,.T.);
#61341=ORIENTED_EDGE('',*,*,#46008,.T.);
#61342=ORIENTED_EDGE('',*,*,#46009,.T.);
#61343=ORIENTED_EDGE('',*,*,#46010,.T.);
#61344=ORIENTED_EDGE('',*,*,#46011,.T.);
#61345=ORIENTED_EDGE('',*,*,#46012,.T.);
#61346=ORIENTED_EDGE('',*,*,#46013,.T.);
#61347=ORIENTED_EDGE('',*,*,#46014,.T.);
#61348=ORIENTED_EDGE('',*,*,#46015,.T.);
#61349=ORIENTED_EDGE('',*,*,#46016,.T.);
#61350=ORIENTED_EDGE('',*,*,#46017,.T.);
#61351=ORIENTED_EDGE('',*,*,#46018,.T.);
#61352=ORIENTED_EDGE('',*,*,#46019,.T.);
#61353=ORIENTED_EDGE('',*,*,#46020,.T.);
#61354=ORIENTED_EDGE('',*,*,#46021,.T.);
#61355=ORIENTED_EDGE('',*,*,#46022,.T.);
#61356=ORIENTED_EDGE('',*,*,#46023,.T.);
#61357=ORIENTED_EDGE('',*,*,#46024,.T.);
#61358=ORIENTED_EDGE('',*,*,#46025,.T.);
#61359=ORIENTED_EDGE('',*,*,#46026,.T.);
#61360=ORIENTED_EDGE('',*,*,#46027,.T.);
#61361=ORIENTED_EDGE('',*,*,#46028,.T.);
#61362=ORIENTED_EDGE('',*,*,#46029,.T.);
#61363=ORIENTED_EDGE('',*,*,#46030,.T.);
#61364=ORIENTED_EDGE('',*,*,#46031,.T.);
#61365=ORIENTED_EDGE('',*,*,#46032,.T.);
#61366=ORIENTED_EDGE('',*,*,#46033,.T.);
#61367=ORIENTED_EDGE('',*,*,#46034,.T.);
#61368=ORIENTED_EDGE('',*,*,#46035,.T.);
#61369=ORIENTED_EDGE('',*,*,#46036,.T.);
#61370=ORIENTED_EDGE('',*,*,#46037,.T.);
#61371=ORIENTED_EDGE('',*,*,#46038,.T.);
#61372=ORIENTED_EDGE('',*,*,#46039,.T.);
#61373=ORIENTED_EDGE('',*,*,#46040,.T.);
#61374=ORIENTED_EDGE('',*,*,#46041,.T.);
#61375=ORIENTED_EDGE('',*,*,#46042,.T.);
#61376=ORIENTED_EDGE('',*,*,#46043,.T.);
#61377=ORIENTED_EDGE('',*,*,#46044,.T.);
#61378=ORIENTED_EDGE('',*,*,#46045,.T.);
#61379=ORIENTED_EDGE('',*,*,#46046,.T.);
#61380=ORIENTED_EDGE('',*,*,#46047,.T.);
#61381=ORIENTED_EDGE('',*,*,#46048,.T.);
#61382=ORIENTED_EDGE('',*,*,#46049,.T.);
#61383=ORIENTED_EDGE('',*,*,#46050,.T.);
#61384=ORIENTED_EDGE('',*,*,#46051,.T.);
#61385=ORIENTED_EDGE('',*,*,#46052,.T.);
#61386=ORIENTED_EDGE('',*,*,#46053,.T.);
#61387=ORIENTED_EDGE('',*,*,#46054,.T.);
#61388=ORIENTED_EDGE('',*,*,#46055,.T.);
#61389=ORIENTED_EDGE('',*,*,#46056,.T.);
#61390=ORIENTED_EDGE('',*,*,#46057,.T.);
#61391=ORIENTED_EDGE('',*,*,#46058,.T.);
#61392=ORIENTED_EDGE('',*,*,#46059,.T.);
#61393=ORIENTED_EDGE('',*,*,#46060,.T.);
#61394=ORIENTED_EDGE('',*,*,#46061,.T.);
#61395=ORIENTED_EDGE('',*,*,#46062,.T.);
#61396=ORIENTED_EDGE('',*,*,#46063,.T.);
#61397=ORIENTED_EDGE('',*,*,#46064,.T.);
#61398=ORIENTED_EDGE('',*,*,#46065,.T.);
#61399=ORIENTED_EDGE('',*,*,#46066,.T.);
#61400=ORIENTED_EDGE('',*,*,#46067,.T.);
#61401=ORIENTED_EDGE('',*,*,#46068,.T.);
#61402=ORIENTED_EDGE('',*,*,#46069,.T.);
#61403=ORIENTED_EDGE('',*,*,#46070,.T.);
#61404=ORIENTED_EDGE('',*,*,#46071,.T.);
#61405=ORIENTED_EDGE('',*,*,#46072,.T.);
#61406=ORIENTED_EDGE('',*,*,#46073,.T.);
#61407=ORIENTED_EDGE('',*,*,#46074,.T.);
#61408=ORIENTED_EDGE('',*,*,#46075,.T.);
#61409=ORIENTED_EDGE('',*,*,#46076,.T.);
#61410=ORIENTED_EDGE('',*,*,#46077,.T.);
#61411=ORIENTED_EDGE('',*,*,#46078,.T.);
#61412=ORIENTED_EDGE('',*,*,#46079,.T.);
#61413=ORIENTED_EDGE('',*,*,#46080,.T.);
#61414=ORIENTED_EDGE('',*,*,#46081,.T.);
#61415=ORIENTED_EDGE('',*,*,#46082,.T.);
#61416=ORIENTED_EDGE('',*,*,#46083,.T.);
#61417=ORIENTED_EDGE('',*,*,#46084,.T.);
#61418=ORIENTED_EDGE('',*,*,#46085,.T.);
#61419=ORIENTED_EDGE('',*,*,#46086,.T.);
#61420=ORIENTED_EDGE('',*,*,#46087,.T.);
#61421=ORIENTED_EDGE('',*,*,#46088,.T.);
#61422=ORIENTED_EDGE('',*,*,#46089,.T.);
#61423=ORIENTED_EDGE('',*,*,#46090,.T.);
#61424=ORIENTED_EDGE('',*,*,#46091,.T.);
#61425=ORIENTED_EDGE('',*,*,#46092,.T.);
#61426=ORIENTED_EDGE('',*,*,#46093,.T.);
#61427=ORIENTED_EDGE('',*,*,#46094,.T.);
#61428=ORIENTED_EDGE('',*,*,#46095,.T.);
#61429=ORIENTED_EDGE('',*,*,#46096,.T.);
#61430=ORIENTED_EDGE('',*,*,#45894,.T.);
#61431=ORIENTED_EDGE('',*,*,#46097,.T.);
#61432=ORIENTED_EDGE('',*,*,#45908,.T.);
#61433=ORIENTED_EDGE('',*,*,#45909,.T.);
#61434=ORIENTED_EDGE('',*,*,#46097,.F.);
#61435=ORIENTED_EDGE('',*,*,#45898,.T.);
#61436=ORIENTED_EDGE('',*,*,#46098,.T.);
#61437=ORIENTED_EDGE('',*,*,#46099,.T.);
#61438=ORIENTED_EDGE('',*,*,#46100,.T.);
#61439=ORIENTED_EDGE('',*,*,#46101,.T.);
#61440=ORIENTED_EDGE('',*,*,#46102,.T.);
#61441=ORIENTED_EDGE('',*,*,#46103,.T.);
#61442=ORIENTED_EDGE('',*,*,#46104,.T.);
#61443=ORIENTED_EDGE('',*,*,#46105,.T.);
#61444=ORIENTED_EDGE('',*,*,#46106,.T.);
#61445=ORIENTED_EDGE('',*,*,#46107,.T.);
#61446=ORIENTED_EDGE('',*,*,#46108,.T.);
#61447=ORIENTED_EDGE('',*,*,#46109,.T.);
#61448=ORIENTED_EDGE('',*,*,#46110,.T.);
#61449=ORIENTED_EDGE('',*,*,#46111,.T.);
#61450=ORIENTED_EDGE('',*,*,#46112,.T.);
#61451=ORIENTED_EDGE('',*,*,#46113,.T.);
#61452=ORIENTED_EDGE('',*,*,#46114,.T.);
#61453=ORIENTED_EDGE('',*,*,#46115,.T.);
#61454=ORIENTED_EDGE('',*,*,#46116,.T.);
#61455=ORIENTED_EDGE('',*,*,#46117,.T.);
#61456=ORIENTED_EDGE('',*,*,#46118,.T.);
#61457=ORIENTED_EDGE('',*,*,#46119,.T.);
#61458=ORIENTED_EDGE('',*,*,#46120,.T.);
#61459=ORIENTED_EDGE('',*,*,#46121,.T.);
#61460=ORIENTED_EDGE('',*,*,#46122,.T.);
#61461=ORIENTED_EDGE('',*,*,#46123,.T.);
#61462=ORIENTED_EDGE('',*,*,#46124,.T.);
#61463=ORIENTED_EDGE('',*,*,#46125,.T.);
#61464=ORIENTED_EDGE('',*,*,#46126,.T.);
#61465=ORIENTED_EDGE('',*,*,#46127,.T.);
#61466=ORIENTED_EDGE('',*,*,#46128,.T.);
#61467=ORIENTED_EDGE('',*,*,#46129,.T.);
#61468=ORIENTED_EDGE('',*,*,#46130,.T.);
#61469=ORIENTED_EDGE('',*,*,#46131,.T.);
#61470=ORIENTED_EDGE('',*,*,#46132,.T.);
#61471=ORIENTED_EDGE('',*,*,#46133,.T.);
#61472=ORIENTED_EDGE('',*,*,#46134,.T.);
#61473=ORIENTED_EDGE('',*,*,#46135,.T.);
#61474=ORIENTED_EDGE('',*,*,#46136,.T.);
#61475=ORIENTED_EDGE('',*,*,#46137,.T.);
#61476=ORIENTED_EDGE('',*,*,#46138,.T.);
#61477=ORIENTED_EDGE('',*,*,#46139,.T.);
#61478=ORIENTED_EDGE('',*,*,#46140,.T.);
#61479=ORIENTED_EDGE('',*,*,#46141,.T.);
#61480=ORIENTED_EDGE('',*,*,#46142,.T.);
#61481=ORIENTED_EDGE('',*,*,#46143,.T.);
#61482=ORIENTED_EDGE('',*,*,#46144,.T.);
#61483=ORIENTED_EDGE('',*,*,#46145,.T.);
#61484=ORIENTED_EDGE('',*,*,#46146,.T.);
#61485=ORIENTED_EDGE('',*,*,#46147,.T.);
#61486=ORIENTED_EDGE('',*,*,#46148,.T.);
#61487=ORIENTED_EDGE('',*,*,#46149,.T.);
#61488=ORIENTED_EDGE('',*,*,#46150,.T.);
#61489=ORIENTED_EDGE('',*,*,#46151,.T.);
#61490=ORIENTED_EDGE('',*,*,#46152,.T.);
#61491=ORIENTED_EDGE('',*,*,#46153,.T.);
#61492=ORIENTED_EDGE('',*,*,#46154,.T.);
#61493=ORIENTED_EDGE('',*,*,#46155,.T.);
#61494=ORIENTED_EDGE('',*,*,#46156,.T.);
#61495=ORIENTED_EDGE('',*,*,#46157,.T.);
#61496=ORIENTED_EDGE('',*,*,#46158,.T.);
#61497=ORIENTED_EDGE('',*,*,#46159,.T.);
#61498=ORIENTED_EDGE('',*,*,#46160,.T.);
#61499=ORIENTED_EDGE('',*,*,#46161,.T.);
#61500=ORIENTED_EDGE('',*,*,#46162,.T.);
#61501=ORIENTED_EDGE('',*,*,#46163,.T.);
#61502=ORIENTED_EDGE('',*,*,#46164,.T.);
#61503=ORIENTED_EDGE('',*,*,#46165,.T.);
#61504=ORIENTED_EDGE('',*,*,#46166,.T.);
#61505=ORIENTED_EDGE('',*,*,#46167,.T.);
#61506=ORIENTED_EDGE('',*,*,#46168,.T.);
#61507=ORIENTED_EDGE('',*,*,#46169,.T.);
#61508=ORIENTED_EDGE('',*,*,#46170,.T.);
#61509=ORIENTED_EDGE('',*,*,#46171,.T.);
#61510=ORIENTED_EDGE('',*,*,#46172,.T.);
#61511=ORIENTED_EDGE('',*,*,#46173,.T.);
#61512=ORIENTED_EDGE('',*,*,#46174,.T.);
#61513=ORIENTED_EDGE('',*,*,#46175,.T.);
#61514=ORIENTED_EDGE('',*,*,#46176,.T.);
#61515=ORIENTED_EDGE('',*,*,#46177,.T.);
#61516=ORIENTED_EDGE('',*,*,#46178,.T.);
#61517=ORIENTED_EDGE('',*,*,#46179,.T.);
#61518=ORIENTED_EDGE('',*,*,#46180,.T.);
#61519=ORIENTED_EDGE('',*,*,#46181,.T.);
#61520=ORIENTED_EDGE('',*,*,#46182,.T.);
#61521=ORIENTED_EDGE('',*,*,#46183,.T.);
#61522=ORIENTED_EDGE('',*,*,#46184,.T.);
#61523=ORIENTED_EDGE('',*,*,#46185,.T.);
#61524=ORIENTED_EDGE('',*,*,#46186,.T.);
#61525=ORIENTED_EDGE('',*,*,#45886,.T.);
#61526=ORIENTED_EDGE('',*,*,#46187,.T.);
#61527=ORIENTED_EDGE('',*,*,#46188,.T.);
#61528=ORIENTED_EDGE('',*,*,#46189,.T.);
#61529=ORIENTED_EDGE('',*,*,#46190,.T.);
#61530=ORIENTED_EDGE('',*,*,#46191,.T.);
#61531=ORIENTED_EDGE('',*,*,#46192,.T.);
#61532=ORIENTED_EDGE('',*,*,#46193,.T.);
#61533=ORIENTED_EDGE('',*,*,#46194,.T.);
#61534=ORIENTED_EDGE('',*,*,#46195,.T.);
#61535=ORIENTED_EDGE('',*,*,#46196,.T.);
#61536=ORIENTED_EDGE('',*,*,#46197,.T.);
#61537=ORIENTED_EDGE('',*,*,#46198,.T.);
#61538=ORIENTED_EDGE('',*,*,#46199,.T.);
#61539=ORIENTED_EDGE('',*,*,#46200,.T.);
#61540=ORIENTED_EDGE('',*,*,#46201,.T.);
#61541=ORIENTED_EDGE('',*,*,#46202,.T.);
#61542=ORIENTED_EDGE('',*,*,#46203,.T.);
#61543=ORIENTED_EDGE('',*,*,#46204,.T.);
#61544=ORIENTED_EDGE('',*,*,#46205,.T.);
#61545=ORIENTED_EDGE('',*,*,#46206,.T.);
#61546=ORIENTED_EDGE('',*,*,#46207,.T.);
#61547=ORIENTED_EDGE('',*,*,#46208,.T.);
#61548=ORIENTED_EDGE('',*,*,#46209,.T.);
#61549=ORIENTED_EDGE('',*,*,#46210,.T.);
#61550=ORIENTED_EDGE('',*,*,#46211,.T.);
#61551=ORIENTED_EDGE('',*,*,#46212,.T.);
#61552=ORIENTED_EDGE('',*,*,#46213,.T.);
#61553=ORIENTED_EDGE('',*,*,#46214,.T.);
#61554=ORIENTED_EDGE('',*,*,#46215,.T.);
#61555=ORIENTED_EDGE('',*,*,#46216,.T.);
#61556=ORIENTED_EDGE('',*,*,#46217,.T.);
#61557=ORIENTED_EDGE('',*,*,#46218,.T.);
#61558=ORIENTED_EDGE('',*,*,#46219,.T.);
#61559=ORIENTED_EDGE('',*,*,#46220,.T.);
#61560=ORIENTED_EDGE('',*,*,#46221,.T.);
#61561=ORIENTED_EDGE('',*,*,#46222,.T.);
#61562=ORIENTED_EDGE('',*,*,#46223,.T.);
#61563=ORIENTED_EDGE('',*,*,#46224,.T.);
#61564=ORIENTED_EDGE('',*,*,#46225,.T.);
#61565=ORIENTED_EDGE('',*,*,#46226,.T.);
#61566=ORIENTED_EDGE('',*,*,#46227,.T.);
#61567=ORIENTED_EDGE('',*,*,#46228,.T.);
#61568=ORIENTED_EDGE('',*,*,#46229,.T.);
#61569=ORIENTED_EDGE('',*,*,#46230,.T.);
#61570=ORIENTED_EDGE('',*,*,#46231,.T.);
#61571=ORIENTED_EDGE('',*,*,#46232,.T.);
#61572=ORIENTED_EDGE('',*,*,#46233,.T.);
#61573=ORIENTED_EDGE('',*,*,#46234,.T.);
#61574=ORIENTED_EDGE('',*,*,#46235,.T.);
#61575=ORIENTED_EDGE('',*,*,#46236,.T.);
#61576=ORIENTED_EDGE('',*,*,#46237,.T.);
#61577=ORIENTED_EDGE('',*,*,#46238,.T.);
#61578=ORIENTED_EDGE('',*,*,#46239,.T.);
#61579=ORIENTED_EDGE('',*,*,#46240,.T.);
#61580=ORIENTED_EDGE('',*,*,#46241,.T.);
#61581=ORIENTED_EDGE('',*,*,#46242,.T.);
#61582=ORIENTED_EDGE('',*,*,#46243,.T.);
#61583=ORIENTED_EDGE('',*,*,#46244,.T.);
#61584=ORIENTED_EDGE('',*,*,#46245,.T.);
#61585=ORIENTED_EDGE('',*,*,#46246,.T.);
#61586=ORIENTED_EDGE('',*,*,#46247,.T.);
#61587=ORIENTED_EDGE('',*,*,#46248,.T.);
#61588=ORIENTED_EDGE('',*,*,#46249,.T.);
#61589=ORIENTED_EDGE('',*,*,#46250,.T.);
#61590=ORIENTED_EDGE('',*,*,#46251,.T.);
#61591=ORIENTED_EDGE('',*,*,#46252,.T.);
#61592=ORIENTED_EDGE('',*,*,#46253,.T.);
#61593=ORIENTED_EDGE('',*,*,#46254,.T.);
#61594=ORIENTED_EDGE('',*,*,#46255,.T.);
#61595=ORIENTED_EDGE('',*,*,#46256,.T.);
#61596=ORIENTED_EDGE('',*,*,#46257,.T.);
#61597=ORIENTED_EDGE('',*,*,#46258,.T.);
#61598=ORIENTED_EDGE('',*,*,#46259,.T.);
#61599=ORIENTED_EDGE('',*,*,#46260,.T.);
#61600=ORIENTED_EDGE('',*,*,#46261,.T.);
#61601=ORIENTED_EDGE('',*,*,#46262,.T.);
#61602=ORIENTED_EDGE('',*,*,#46263,.T.);
#61603=ORIENTED_EDGE('',*,*,#46264,.T.);
#61604=ORIENTED_EDGE('',*,*,#46265,.T.);
#61605=ORIENTED_EDGE('',*,*,#46266,.T.);
#61606=ORIENTED_EDGE('',*,*,#46267,.T.);
#61607=ORIENTED_EDGE('',*,*,#46268,.T.);
#61608=ORIENTED_EDGE('',*,*,#46269,.T.);
#61609=ORIENTED_EDGE('',*,*,#46270,.T.);
#61610=ORIENTED_EDGE('',*,*,#46271,.T.);
#61611=ORIENTED_EDGE('',*,*,#46272,.T.);
#61612=ORIENTED_EDGE('',*,*,#46273,.T.);
#61613=ORIENTED_EDGE('',*,*,#46274,.T.);
#61614=ORIENTED_EDGE('',*,*,#46275,.T.);
#61615=ORIENTED_EDGE('',*,*,#45892,.T.);
#61616=ORIENTED_EDGE('',*,*,#46276,.T.);
#61617=ORIENTED_EDGE('',*,*,#46277,.T.);
#61618=ORIENTED_EDGE('',*,*,#46278,.T.);
#61619=ORIENTED_EDGE('',*,*,#46279,.T.);
#61620=ORIENTED_EDGE('',*,*,#46280,.T.);
#61621=ORIENTED_EDGE('',*,*,#46281,.T.);
#61622=ORIENTED_EDGE('',*,*,#46282,.T.);
#61623=ORIENTED_EDGE('',*,*,#46283,.T.);
#61624=ORIENTED_EDGE('',*,*,#46284,.T.);
#61625=ORIENTED_EDGE('',*,*,#46285,.T.);
#61626=ORIENTED_EDGE('',*,*,#46286,.T.);
#61627=ORIENTED_EDGE('',*,*,#46287,.T.);
#61628=ORIENTED_EDGE('',*,*,#46288,.T.);
#61629=ORIENTED_EDGE('',*,*,#46289,.T.);
#61630=ORIENTED_EDGE('',*,*,#46290,.T.);
#61631=ORIENTED_EDGE('',*,*,#46291,.T.);
#61632=ORIENTED_EDGE('',*,*,#46292,.T.);
#61633=ORIENTED_EDGE('',*,*,#46293,.T.);
#61634=ORIENTED_EDGE('',*,*,#46294,.T.);
#61635=ORIENTED_EDGE('',*,*,#46295,.T.);
#61636=ORIENTED_EDGE('',*,*,#46296,.T.);
#61637=ORIENTED_EDGE('',*,*,#46297,.T.);
#61638=ORIENTED_EDGE('',*,*,#46298,.T.);
#61639=ORIENTED_EDGE('',*,*,#46299,.T.);
#61640=ORIENTED_EDGE('',*,*,#46300,.T.);
#61641=ORIENTED_EDGE('',*,*,#46301,.T.);
#61642=ORIENTED_EDGE('',*,*,#46302,.T.);
#61643=ORIENTED_EDGE('',*,*,#46303,.T.);
#61644=ORIENTED_EDGE('',*,*,#46304,.T.);
#61645=ORIENTED_EDGE('',*,*,#46305,.T.);
#61646=ORIENTED_EDGE('',*,*,#46306,.T.);
#61647=ORIENTED_EDGE('',*,*,#46307,.T.);
#61648=ORIENTED_EDGE('',*,*,#46308,.T.);
#61649=ORIENTED_EDGE('',*,*,#46309,.T.);
#61650=ORIENTED_EDGE('',*,*,#46310,.T.);
#61651=ORIENTED_EDGE('',*,*,#46311,.T.);
#61652=ORIENTED_EDGE('',*,*,#46312,.T.);
#61653=ORIENTED_EDGE('',*,*,#46313,.T.);
#61654=ORIENTED_EDGE('',*,*,#46314,.T.);
#61655=ORIENTED_EDGE('',*,*,#46315,.T.);
#61656=ORIENTED_EDGE('',*,*,#46316,.T.);
#61657=ORIENTED_EDGE('',*,*,#46317,.T.);
#61658=ORIENTED_EDGE('',*,*,#46318,.T.);
#61659=ORIENTED_EDGE('',*,*,#46319,.T.);
#61660=ORIENTED_EDGE('',*,*,#46320,.T.);
#61661=ORIENTED_EDGE('',*,*,#46321,.T.);
#61662=ORIENTED_EDGE('',*,*,#46322,.T.);
#61663=ORIENTED_EDGE('',*,*,#46323,.T.);
#61664=ORIENTED_EDGE('',*,*,#46324,.T.);
#61665=ORIENTED_EDGE('',*,*,#46325,.T.);
#61666=ORIENTED_EDGE('',*,*,#46326,.T.);
#61667=ORIENTED_EDGE('',*,*,#46327,.T.);
#61668=ORIENTED_EDGE('',*,*,#46328,.T.);
#61669=ORIENTED_EDGE('',*,*,#46329,.T.);
#61670=ORIENTED_EDGE('',*,*,#46330,.T.);
#61671=ORIENTED_EDGE('',*,*,#46331,.T.);
#61672=ORIENTED_EDGE('',*,*,#46332,.T.);
#61673=ORIENTED_EDGE('',*,*,#46333,.T.);
#61674=ORIENTED_EDGE('',*,*,#46334,.T.);
#61675=ORIENTED_EDGE('',*,*,#46335,.T.);
#61676=ORIENTED_EDGE('',*,*,#46336,.T.);
#61677=ORIENTED_EDGE('',*,*,#46337,.T.);
#61678=ORIENTED_EDGE('',*,*,#46338,.T.);
#61679=ORIENTED_EDGE('',*,*,#46339,.T.);
#61680=ORIENTED_EDGE('',*,*,#46340,.T.);
#61681=ORIENTED_EDGE('',*,*,#46341,.T.);
#61682=ORIENTED_EDGE('',*,*,#46342,.T.);
#61683=ORIENTED_EDGE('',*,*,#46343,.T.);
#61684=ORIENTED_EDGE('',*,*,#46344,.T.);
#61685=ORIENTED_EDGE('',*,*,#46345,.T.);
#61686=ORIENTED_EDGE('',*,*,#46346,.T.);
#61687=ORIENTED_EDGE('',*,*,#46347,.T.);
#61688=ORIENTED_EDGE('',*,*,#46348,.T.);
#61689=ORIENTED_EDGE('',*,*,#46349,.T.);
#61690=ORIENTED_EDGE('',*,*,#46350,.T.);
#61691=ORIENTED_EDGE('',*,*,#46351,.T.);
#61692=ORIENTED_EDGE('',*,*,#46352,.T.);
#61693=ORIENTED_EDGE('',*,*,#46353,.T.);
#61694=ORIENTED_EDGE('',*,*,#46354,.T.);
#61695=ORIENTED_EDGE('',*,*,#46355,.T.);
#61696=ORIENTED_EDGE('',*,*,#46356,.T.);
#61697=ORIENTED_EDGE('',*,*,#46357,.T.);
#61698=ORIENTED_EDGE('',*,*,#46358,.T.);
#61699=ORIENTED_EDGE('',*,*,#46359,.T.);
#61700=ORIENTED_EDGE('',*,*,#46360,.T.);
#61701=ORIENTED_EDGE('',*,*,#46361,.T.);
#61702=ORIENTED_EDGE('',*,*,#46362,.T.);
#61703=ORIENTED_EDGE('',*,*,#46363,.T.);
#61704=ORIENTED_EDGE('',*,*,#46364,.T.);
#61705=ORIENTED_EDGE('',*,*,#46365,.T.);
#61706=ORIENTED_EDGE('',*,*,#46366,.T.);
#61707=ORIENTED_EDGE('',*,*,#46367,.T.);
#61708=ORIENTED_EDGE('',*,*,#46368,.T.);
#61709=ORIENTED_EDGE('',*,*,#46369,.T.);
#61710=ORIENTED_EDGE('',*,*,#46370,.T.);
#61711=ORIENTED_EDGE('',*,*,#46371,.T.);
#61712=ORIENTED_EDGE('',*,*,#46372,.T.);
#61713=ORIENTED_EDGE('',*,*,#46373,.T.);
#61714=ORIENTED_EDGE('',*,*,#46374,.T.);
#61715=ORIENTED_EDGE('',*,*,#46375,.T.);
#61716=ORIENTED_EDGE('',*,*,#46376,.T.);
#61717=ORIENTED_EDGE('',*,*,#46377,.T.);
#61718=ORIENTED_EDGE('',*,*,#46378,.T.);
#61719=ORIENTED_EDGE('',*,*,#46379,.T.);
#61720=ORIENTED_EDGE('',*,*,#46380,.T.);
#61721=ORIENTED_EDGE('',*,*,#46381,.T.);
#61722=ORIENTED_EDGE('',*,*,#46382,.T.);
#61723=ORIENTED_EDGE('',*,*,#46383,.T.);
#61724=ORIENTED_EDGE('',*,*,#46384,.T.);
#61725=ORIENTED_EDGE('',*,*,#46385,.T.);
#61726=ORIENTED_EDGE('',*,*,#46386,.T.);
#61727=ORIENTED_EDGE('',*,*,#46387,.T.);
#61728=ORIENTED_EDGE('',*,*,#46388,.T.);
#61729=ORIENTED_EDGE('',*,*,#46389,.T.);
#61730=ORIENTED_EDGE('',*,*,#46390,.T.);
#61731=ORIENTED_EDGE('',*,*,#46391,.T.);
#61732=ORIENTED_EDGE('',*,*,#46392,.T.);
#61733=ORIENTED_EDGE('',*,*,#46393,.T.);
#61734=ORIENTED_EDGE('',*,*,#46394,.T.);
#61735=ORIENTED_EDGE('',*,*,#46395,.T.);
#61736=ORIENTED_EDGE('',*,*,#46396,.T.);
#61737=ORIENTED_EDGE('',*,*,#46397,.T.);
#61738=ORIENTED_EDGE('',*,*,#46398,.T.);
#61739=ORIENTED_EDGE('',*,*,#46399,.T.);
#61740=ORIENTED_EDGE('',*,*,#46400,.T.);
#61741=ORIENTED_EDGE('',*,*,#46401,.T.);
#61742=ORIENTED_EDGE('',*,*,#46402,.T.);
#61743=ORIENTED_EDGE('',*,*,#46403,.T.);
#61744=ORIENTED_EDGE('',*,*,#46404,.T.);
#61745=ORIENTED_EDGE('',*,*,#46405,.T.);
#61746=ORIENTED_EDGE('',*,*,#46406,.T.);
#61747=ORIENTED_EDGE('',*,*,#46407,.T.);
#61748=ORIENTED_EDGE('',*,*,#46408,.T.);
#61749=ORIENTED_EDGE('',*,*,#46409,.T.);
#61750=ORIENTED_EDGE('',*,*,#46410,.T.);
#61751=ORIENTED_EDGE('',*,*,#46411,.T.);
#61752=ORIENTED_EDGE('',*,*,#46412,.T.);
#61753=ORIENTED_EDGE('',*,*,#46413,.T.);
#61754=ORIENTED_EDGE('',*,*,#46414,.T.);
#61755=ORIENTED_EDGE('',*,*,#46415,.T.);
#61756=ORIENTED_EDGE('',*,*,#46416,.T.);
#61757=ORIENTED_EDGE('',*,*,#46417,.T.);
#61758=ORIENTED_EDGE('',*,*,#46418,.T.);
#61759=ORIENTED_EDGE('',*,*,#46419,.T.);
#61760=ORIENTED_EDGE('',*,*,#46420,.T.);
#61761=ORIENTED_EDGE('',*,*,#46421,.T.);
#61762=ORIENTED_EDGE('',*,*,#46422,.T.);
#61763=ORIENTED_EDGE('',*,*,#46423,.T.);
#61764=ORIENTED_EDGE('',*,*,#46424,.T.);
#61765=ORIENTED_EDGE('',*,*,#46425,.T.);
#61766=ORIENTED_EDGE('',*,*,#46426,.T.);
#61767=ORIENTED_EDGE('',*,*,#46427,.T.);
#61768=ORIENTED_EDGE('',*,*,#46428,.T.);
#61769=ORIENTED_EDGE('',*,*,#46429,.T.);
#61770=ORIENTED_EDGE('',*,*,#46430,.T.);
#61771=ORIENTED_EDGE('',*,*,#46431,.T.);
#61772=ORIENTED_EDGE('',*,*,#46432,.T.);
#61773=ORIENTED_EDGE('',*,*,#46433,.T.);
#61774=ORIENTED_EDGE('',*,*,#46434,.T.);
#61775=ORIENTED_EDGE('',*,*,#46435,.T.);
#61776=ORIENTED_EDGE('',*,*,#46436,.T.);
#61777=ORIENTED_EDGE('',*,*,#46437,.T.);
#61778=ORIENTED_EDGE('',*,*,#46438,.T.);
#61779=ORIENTED_EDGE('',*,*,#46439,.T.);
#61780=ORIENTED_EDGE('',*,*,#46440,.T.);
#61781=ORIENTED_EDGE('',*,*,#46441,.T.);
#61782=ORIENTED_EDGE('',*,*,#46442,.T.);
#61783=ORIENTED_EDGE('',*,*,#46443,.T.);
#61784=ORIENTED_EDGE('',*,*,#46444,.T.);
#61785=ORIENTED_EDGE('',*,*,#46445,.T.);
#61786=ORIENTED_EDGE('',*,*,#46446,.T.);
#61787=ORIENTED_EDGE('',*,*,#46447,.T.);
#61788=ORIENTED_EDGE('',*,*,#46448,.T.);
#61789=ORIENTED_EDGE('',*,*,#46449,.T.);
#61790=ORIENTED_EDGE('',*,*,#46450,.T.);
#61791=ORIENTED_EDGE('',*,*,#46451,.T.);
#61792=ORIENTED_EDGE('',*,*,#46452,.T.);
#61793=ORIENTED_EDGE('',*,*,#46453,.T.);
#61794=ORIENTED_EDGE('',*,*,#46454,.T.);
#61795=ORIENTED_EDGE('',*,*,#46455,.T.);
#61796=ORIENTED_EDGE('',*,*,#46456,.T.);
#61797=ORIENTED_EDGE('',*,*,#45903,.T.);
#61798=ORIENTED_EDGE('',*,*,#46456,.F.);
#61799=ORIENTED_EDGE('',*,*,#46457,.T.);
#61800=ORIENTED_EDGE('',*,*,#46458,.T.);
#61801=ORIENTED_EDGE('',*,*,#46459,.T.);
#61802=ORIENTED_EDGE('',*,*,#46460,.T.);
#61803=ORIENTED_EDGE('',*,*,#46461,.T.);
#61804=ORIENTED_EDGE('',*,*,#46462,.T.);
#61805=ORIENTED_EDGE('',*,*,#46463,.T.);
#61806=ORIENTED_EDGE('',*,*,#46464,.T.);
#61807=ORIENTED_EDGE('',*,*,#46465,.T.);
#61808=ORIENTED_EDGE('',*,*,#46466,.T.);
#61809=ORIENTED_EDGE('',*,*,#46467,.T.);
#61810=ORIENTED_EDGE('',*,*,#46468,.T.);
#61811=ORIENTED_EDGE('',*,*,#46469,.T.);
#61812=ORIENTED_EDGE('',*,*,#46470,.T.);
#61813=ORIENTED_EDGE('',*,*,#46471,.T.);
#61814=ORIENTED_EDGE('',*,*,#46472,.T.);
#61815=ORIENTED_EDGE('',*,*,#46473,.T.);
#61816=ORIENTED_EDGE('',*,*,#46474,.T.);
#61817=ORIENTED_EDGE('',*,*,#46475,.T.);
#61818=ORIENTED_EDGE('',*,*,#46476,.T.);
#61819=ORIENTED_EDGE('',*,*,#46477,.T.);
#61820=ORIENTED_EDGE('',*,*,#46478,.T.);
#61821=ORIENTED_EDGE('',*,*,#46479,.T.);
#61822=ORIENTED_EDGE('',*,*,#46480,.T.);
#61823=ORIENTED_EDGE('',*,*,#46481,.T.);
#61824=ORIENTED_EDGE('',*,*,#46482,.T.);
#61825=ORIENTED_EDGE('',*,*,#46483,.T.);
#61826=ORIENTED_EDGE('',*,*,#46484,.T.);
#61827=ORIENTED_EDGE('',*,*,#46485,.T.);
#61828=ORIENTED_EDGE('',*,*,#46486,.T.);
#61829=ORIENTED_EDGE('',*,*,#46487,.T.);
#61830=ORIENTED_EDGE('',*,*,#46488,.T.);
#61831=ORIENTED_EDGE('',*,*,#46489,.T.);
#61832=ORIENTED_EDGE('',*,*,#46490,.T.);
#61833=ORIENTED_EDGE('',*,*,#46491,.T.);
#61834=ORIENTED_EDGE('',*,*,#46492,.T.);
#61835=ORIENTED_EDGE('',*,*,#46493,.T.);
#61836=ORIENTED_EDGE('',*,*,#46494,.T.);
#61837=ORIENTED_EDGE('',*,*,#46495,.T.);
#61838=ORIENTED_EDGE('',*,*,#46496,.T.);
#61839=ORIENTED_EDGE('',*,*,#46497,.T.);
#61840=ORIENTED_EDGE('',*,*,#46498,.T.);
#61841=ORIENTED_EDGE('',*,*,#46499,.T.);
#61842=ORIENTED_EDGE('',*,*,#46500,.T.);
#61843=ORIENTED_EDGE('',*,*,#46501,.T.);
#61844=ORIENTED_EDGE('',*,*,#46502,.T.);
#61845=ORIENTED_EDGE('',*,*,#46503,.T.);
#61846=ORIENTED_EDGE('',*,*,#46504,.T.);
#61847=ORIENTED_EDGE('',*,*,#46505,.T.);
#61848=ORIENTED_EDGE('',*,*,#46506,.T.);
#61849=ORIENTED_EDGE('',*,*,#46507,.T.);
#61850=ORIENTED_EDGE('',*,*,#46508,.T.);
#61851=ORIENTED_EDGE('',*,*,#46509,.T.);
#61852=ORIENTED_EDGE('',*,*,#46510,.T.);
#61853=ORIENTED_EDGE('',*,*,#46511,.T.);
#61854=ORIENTED_EDGE('',*,*,#46512,.T.);
#61855=ORIENTED_EDGE('',*,*,#46513,.T.);
#61856=ORIENTED_EDGE('',*,*,#46514,.T.);
#61857=ORIENTED_EDGE('',*,*,#46515,.T.);
#61858=ORIENTED_EDGE('',*,*,#46516,.T.);
#61859=ORIENTED_EDGE('',*,*,#46517,.T.);
#61860=ORIENTED_EDGE('',*,*,#46518,.T.);
#61861=ORIENTED_EDGE('',*,*,#46519,.T.);
#61862=ORIENTED_EDGE('',*,*,#46520,.T.);
#61863=ORIENTED_EDGE('',*,*,#46521,.T.);
#61864=ORIENTED_EDGE('',*,*,#46522,.T.);
#61865=ORIENTED_EDGE('',*,*,#46523,.T.);
#61866=ORIENTED_EDGE('',*,*,#46524,.T.);
#61867=ORIENTED_EDGE('',*,*,#46525,.T.);
#61868=ORIENTED_EDGE('',*,*,#46526,.T.);
#61869=ORIENTED_EDGE('',*,*,#46527,.T.);
#61870=ORIENTED_EDGE('',*,*,#46528,.T.);
#61871=ORIENTED_EDGE('',*,*,#46529,.T.);
#61872=ORIENTED_EDGE('',*,*,#46530,.T.);
#61873=ORIENTED_EDGE('',*,*,#46531,.T.);
#61874=ORIENTED_EDGE('',*,*,#46532,.T.);
#61875=ORIENTED_EDGE('',*,*,#46533,.T.);
#61876=ORIENTED_EDGE('',*,*,#46534,.T.);
#61877=ORIENTED_EDGE('',*,*,#46535,.T.);
#61878=ORIENTED_EDGE('',*,*,#46536,.T.);
#61879=ORIENTED_EDGE('',*,*,#46537,.T.);
#61880=ORIENTED_EDGE('',*,*,#46538,.T.);
#61881=ORIENTED_EDGE('',*,*,#46539,.T.);
#61882=ORIENTED_EDGE('',*,*,#46540,.T.);
#61883=ORIENTED_EDGE('',*,*,#46541,.T.);
#61884=ORIENTED_EDGE('',*,*,#46542,.T.);
#61885=ORIENTED_EDGE('',*,*,#46543,.T.);
#61886=ORIENTED_EDGE('',*,*,#46544,.T.);
#61887=ORIENTED_EDGE('',*,*,#46545,.T.);
#61888=ORIENTED_EDGE('',*,*,#46546,.T.);
#61889=ORIENTED_EDGE('',*,*,#45884,.T.);
#61890=ORIENTED_EDGE('',*,*,#46547,.T.);
#61891=ORIENTED_EDGE('',*,*,#46548,.T.);
#61892=ORIENTED_EDGE('',*,*,#46549,.T.);
#61893=ORIENTED_EDGE('',*,*,#46550,.T.);
#61894=ORIENTED_EDGE('',*,*,#46551,.T.);
#61895=ORIENTED_EDGE('',*,*,#46552,.T.);
#61896=ORIENTED_EDGE('',*,*,#46553,.T.);
#61897=ORIENTED_EDGE('',*,*,#46554,.T.);
#61898=ORIENTED_EDGE('',*,*,#46555,.T.);
#61899=ORIENTED_EDGE('',*,*,#46556,.T.);
#61900=ORIENTED_EDGE('',*,*,#46557,.T.);
#61901=ORIENTED_EDGE('',*,*,#46558,.T.);
#61902=ORIENTED_EDGE('',*,*,#46559,.T.);
#61903=ORIENTED_EDGE('',*,*,#46560,.T.);
#61904=ORIENTED_EDGE('',*,*,#46561,.T.);
#61905=ORIENTED_EDGE('',*,*,#46562,.T.);
#61906=ORIENTED_EDGE('',*,*,#46563,.T.);
#61907=ORIENTED_EDGE('',*,*,#46564,.T.);
#61908=ORIENTED_EDGE('',*,*,#46565,.T.);
#61909=ORIENTED_EDGE('',*,*,#46566,.T.);
#61910=ORIENTED_EDGE('',*,*,#46567,.T.);
#61911=ORIENTED_EDGE('',*,*,#46568,.T.);
#61912=ORIENTED_EDGE('',*,*,#46569,.T.);
#61913=ORIENTED_EDGE('',*,*,#46570,.T.);
#61914=ORIENTED_EDGE('',*,*,#46571,.T.);
#61915=ORIENTED_EDGE('',*,*,#46572,.T.);
#61916=ORIENTED_EDGE('',*,*,#46573,.T.);
#61917=ORIENTED_EDGE('',*,*,#46574,.T.);
#61918=ORIENTED_EDGE('',*,*,#46575,.T.);
#61919=ORIENTED_EDGE('',*,*,#46576,.T.);
#61920=ORIENTED_EDGE('',*,*,#46577,.T.);
#61921=ORIENTED_EDGE('',*,*,#46578,.T.);
#61922=ORIENTED_EDGE('',*,*,#46579,.T.);
#61923=ORIENTED_EDGE('',*,*,#46580,.T.);
#61924=ORIENTED_EDGE('',*,*,#46581,.T.);
#61925=ORIENTED_EDGE('',*,*,#46582,.T.);
#61926=ORIENTED_EDGE('',*,*,#46583,.T.);
#61927=ORIENTED_EDGE('',*,*,#46584,.T.);
#61928=ORIENTED_EDGE('',*,*,#46585,.T.);
#61929=ORIENTED_EDGE('',*,*,#46586,.T.);
#61930=ORIENTED_EDGE('',*,*,#46587,.T.);
#61931=ORIENTED_EDGE('',*,*,#46588,.T.);
#61932=ORIENTED_EDGE('',*,*,#46589,.T.);
#61933=ORIENTED_EDGE('',*,*,#46590,.T.);
#61934=ORIENTED_EDGE('',*,*,#46591,.T.);
#61935=ORIENTED_EDGE('',*,*,#46592,.T.);
#61936=ORIENTED_EDGE('',*,*,#46593,.T.);
#61937=ORIENTED_EDGE('',*,*,#46594,.T.);
#61938=ORIENTED_EDGE('',*,*,#46595,.T.);
#61939=ORIENTED_EDGE('',*,*,#46596,.T.);
#61940=ORIENTED_EDGE('',*,*,#46597,.T.);
#61941=ORIENTED_EDGE('',*,*,#46598,.T.);
#61942=ORIENTED_EDGE('',*,*,#46599,.T.);
#61943=ORIENTED_EDGE('',*,*,#46600,.T.);
#61944=ORIENTED_EDGE('',*,*,#46601,.T.);
#61945=ORIENTED_EDGE('',*,*,#46602,.T.);
#61946=ORIENTED_EDGE('',*,*,#46603,.T.);
#61947=ORIENTED_EDGE('',*,*,#46604,.T.);
#61948=ORIENTED_EDGE('',*,*,#46605,.T.);
#61949=ORIENTED_EDGE('',*,*,#46606,.T.);
#61950=ORIENTED_EDGE('',*,*,#46607,.T.);
#61951=ORIENTED_EDGE('',*,*,#46608,.T.);
#61952=ORIENTED_EDGE('',*,*,#46609,.T.);
#61953=ORIENTED_EDGE('',*,*,#46610,.T.);
#61954=ORIENTED_EDGE('',*,*,#46611,.T.);
#61955=ORIENTED_EDGE('',*,*,#46612,.T.);
#61956=ORIENTED_EDGE('',*,*,#46613,.T.);
#61957=ORIENTED_EDGE('',*,*,#46614,.T.);
#61958=ORIENTED_EDGE('',*,*,#46615,.T.);
#61959=ORIENTED_EDGE('',*,*,#46616,.T.);
#61960=ORIENTED_EDGE('',*,*,#46617,.T.);
#61961=ORIENTED_EDGE('',*,*,#46618,.T.);
#61962=ORIENTED_EDGE('',*,*,#46619,.T.);
#61963=ORIENTED_EDGE('',*,*,#46620,.T.);
#61964=ORIENTED_EDGE('',*,*,#46621,.T.);
#61965=ORIENTED_EDGE('',*,*,#46622,.T.);
#61966=ORIENTED_EDGE('',*,*,#46623,.T.);
#61967=ORIENTED_EDGE('',*,*,#46624,.T.);
#61968=ORIENTED_EDGE('',*,*,#46625,.T.);
#61969=ORIENTED_EDGE('',*,*,#46626,.T.);
#61970=ORIENTED_EDGE('',*,*,#46627,.T.);
#61971=ORIENTED_EDGE('',*,*,#46628,.T.);
#61972=ORIENTED_EDGE('',*,*,#46629,.T.);
#61973=ORIENTED_EDGE('',*,*,#46630,.T.);
#61974=ORIENTED_EDGE('',*,*,#46631,.T.);
#61975=ORIENTED_EDGE('',*,*,#46632,.T.);
#61976=ORIENTED_EDGE('',*,*,#46633,.T.);
#61977=ORIENTED_EDGE('',*,*,#46634,.T.);
#61978=ORIENTED_EDGE('',*,*,#46635,.T.);
#61979=ORIENTED_EDGE('',*,*,#46636,.T.);
#61980=ORIENTED_EDGE('',*,*,#46637,.T.);
#61981=ORIENTED_EDGE('',*,*,#45901,.T.);
#61982=ORIENTED_EDGE('',*,*,#45902,.T.);
#61983=ORIENTED_EDGE('',*,*,#46637,.F.);
#61984=ORIENTED_EDGE('',*,*,#46638,.T.);
#61985=ORIENTED_EDGE('',*,*,#46636,.F.);
#61986=ORIENTED_EDGE('',*,*,#46639,.T.);
#61987=ORIENTED_EDGE('',*,*,#46640,.T.);
#61988=ORIENTED_EDGE('',*,*,#46639,.F.);
#61989=ORIENTED_EDGE('',*,*,#46638,.F.);
#61990=ORIENTED_EDGE('',*,*,#46641,.F.);
#61991=ORIENTED_EDGE('',*,*,#46642,.T.);
#61992=ORIENTED_EDGE('',*,*,#46643,.T.);
#61993=ORIENTED_EDGE('',*,*,#46644,.T.);
#61994=ORIENTED_EDGE('',*,*,#46645,.F.);
#61995=ORIENTED_EDGE('',*,*,#46646,.F.);
#61996=ORIENTED_EDGE('',*,*,#46647,.T.);
#61997=ORIENTED_EDGE('',*,*,#46648,.T.);
#61998=ORIENTED_EDGE('',*,*,#46646,.T.);
#61999=ORIENTED_EDGE('',*,*,#46649,.T.);
#62000=ORIENTED_EDGE('',*,*,#46650,.T.);
#62001=ORIENTED_EDGE('',*,*,#46651,.T.);
#62002=ORIENTED_EDGE('',*,*,#46652,.T.);
#62003=ORIENTED_EDGE('',*,*,#46653,.T.);
#62004=ORIENTED_EDGE('',*,*,#46654,.F.);
#62005=ORIENTED_EDGE('',*,*,#46655,.T.);
#62006=ORIENTED_EDGE('',*,*,#46656,.T.);
#62007=ORIENTED_EDGE('',*,*,#46657,.T.);
#62008=ORIENTED_EDGE('',*,*,#46658,.F.);
#62009=ORIENTED_EDGE('',*,*,#46659,.F.);
#62010=ORIENTED_EDGE('',*,*,#46660,.T.);
#62011=ORIENTED_EDGE('',*,*,#46661,.T.);
#62012=ORIENTED_EDGE('',*,*,#46659,.T.);
#62013=ORIENTED_EDGE('',*,*,#46662,.T.);
#62014=ORIENTED_EDGE('',*,*,#46643,.F.);
#62015=ORIENTED_EDGE('',*,*,#46663,.T.);
#62016=ORIENTED_EDGE('',*,*,#46460,.F.);
#62017=ORIENTED_EDGE('',*,*,#46664,.T.);
#62018=ORIENTED_EDGE('',*,*,#46273,.F.);
#62019=ORIENTED_EDGE('',*,*,#46665,.T.);
#62020=ORIENTED_EDGE('',*,*,#46660,.F.);
#62021=ORIENTED_EDGE('',*,*,#46666,.T.);
#62022=ORIENTED_EDGE('',*,*,#46656,.F.);
#62023=ORIENTED_EDGE('',*,*,#46667,.T.);
#62024=ORIENTED_EDGE('',*,*,#46650,.F.);
#62025=ORIENTED_EDGE('',*,*,#46668,.T.);
#62026=ORIENTED_EDGE('',*,*,#46652,.F.);
#62027=ORIENTED_EDGE('',*,*,#46669,.T.);
#62028=ORIENTED_EDGE('',*,*,#46647,.F.);
#62029=ORIENTED_EDGE('',*,*,#46670,.T.);
#62030=ORIENTED_EDGE('',*,*,#46671,.T.);
#62031=ORIENTED_EDGE('',*,*,#46672,.T.);
#62032=ORIENTED_EDGE('',*,*,#46673,.F.);
#62033=ORIENTED_EDGE('',*,*,#46674,.F.);
#62034=ORIENTED_EDGE('',*,*,#46675,.F.);
#62035=ORIENTED_EDGE('',*,*,#46676,.T.);
#62036=ORIENTED_EDGE('',*,*,#46674,.T.);
#62037=ORIENTED_EDGE('',*,*,#46677,.T.);
#62038=ORIENTED_EDGE('',*,*,#46678,.T.);
#62039=ORIENTED_EDGE('',*,*,#46679,.T.);
#62040=ORIENTED_EDGE('',*,*,#46680,.T.);
#62041=ORIENTED_EDGE('',*,*,#46681,.T.);
#62042=ORIENTED_EDGE('',*,*,#46682,.T.);
#62043=ORIENTED_EDGE('',*,*,#46683,.T.);
#62044=ORIENTED_EDGE('',*,*,#46684,.T.);
#62045=ORIENTED_EDGE('',*,*,#46685,.T.);
#62046=ORIENTED_EDGE('',*,*,#46686,.F.);
#62047=ORIENTED_EDGE('',*,*,#46687,.F.);
#62048=ORIENTED_EDGE('',*,*,#46688,.F.);
#62049=ORIENTED_EDGE('',*,*,#46689,.T.);
#62050=ORIENTED_EDGE('',*,*,#46687,.T.);
#62051=ORIENTED_EDGE('',*,*,#46690,.T.);
#62052=ORIENTED_EDGE('',*,*,#46691,.T.);
#62053=ORIENTED_EDGE('',*,*,#46692,.T.);
#62054=ORIENTED_EDGE('',*,*,#46466,.F.);
#62055=ORIENTED_EDGE('',*,*,#46693,.T.);
#62056=ORIENTED_EDGE('',*,*,#46671,.F.);
#62057=ORIENTED_EDGE('',*,*,#46694,.T.);
#62058=ORIENTED_EDGE('',*,*,#46691,.F.);
#62059=ORIENTED_EDGE('',*,*,#46695,.T.);
#62060=ORIENTED_EDGE('',*,*,#46267,.F.);
#62061=ORIENTED_EDGE('',*,*,#46696,.T.);
#62062=ORIENTED_EDGE('',*,*,#46682,.F.);
#62063=ORIENTED_EDGE('',*,*,#46697,.T.);
#62064=ORIENTED_EDGE('',*,*,#46684,.F.);
#62065=ORIENTED_EDGE('',*,*,#46698,.T.);
#62066=ORIENTED_EDGE('',*,*,#46678,.F.);
#62067=ORIENTED_EDGE('',*,*,#46699,.T.);
#62068=ORIENTED_EDGE('',*,*,#46680,.F.);
#62069=ORIENTED_EDGE('',*,*,#46700,.T.);
#62070=ORIENTED_EDGE('',*,*,#46701,.T.);
#62071=ORIENTED_EDGE('',*,*,#46702,.T.);
#62072=ORIENTED_EDGE('',*,*,#46703,.F.);
#62073=ORIENTED_EDGE('',*,*,#46704,.F.);
#62074=ORIENTED_EDGE('',*,*,#46705,.F.);
#62075=ORIENTED_EDGE('',*,*,#46706,.T.);
#62076=ORIENTED_EDGE('',*,*,#46704,.T.);
#62077=ORIENTED_EDGE('',*,*,#46707,.T.);
#62078=ORIENTED_EDGE('',*,*,#46708,.T.);
#62079=ORIENTED_EDGE('',*,*,#46709,.T.);
#62080=ORIENTED_EDGE('',*,*,#46710,.T.);
#62081=ORIENTED_EDGE('',*,*,#46711,.T.);
#62082=ORIENTED_EDGE('',*,*,#46712,.T.);
#62083=ORIENTED_EDGE('',*,*,#46713,.T.);
#62084=ORIENTED_EDGE('',*,*,#46714,.T.);
#62085=ORIENTED_EDGE('',*,*,#46715,.T.);
#62086=ORIENTED_EDGE('',*,*,#46716,.F.);
#62087=ORIENTED_EDGE('',*,*,#46717,.F.);
#62088=ORIENTED_EDGE('',*,*,#46718,.F.);
#62089=ORIENTED_EDGE('',*,*,#46719,.T.);
#62090=ORIENTED_EDGE('',*,*,#46717,.T.);
#62091=ORIENTED_EDGE('',*,*,#46720,.T.);
#62092=ORIENTED_EDGE('',*,*,#46721,.T.);
#62093=ORIENTED_EDGE('',*,*,#46722,.T.);
#62094=ORIENTED_EDGE('',*,*,#46472,.F.);
#62095=ORIENTED_EDGE('',*,*,#46723,.T.);
#62096=ORIENTED_EDGE('',*,*,#46701,.F.);
#62097=ORIENTED_EDGE('',*,*,#46724,.T.);
#62098=ORIENTED_EDGE('',*,*,#46721,.F.);
#62099=ORIENTED_EDGE('',*,*,#46725,.T.);
#62100=ORIENTED_EDGE('',*,*,#46261,.F.);
#62101=ORIENTED_EDGE('',*,*,#46726,.T.);
#62102=ORIENTED_EDGE('',*,*,#46712,.F.);
#62103=ORIENTED_EDGE('',*,*,#46727,.T.);
#62104=ORIENTED_EDGE('',*,*,#46714,.F.);
#62105=ORIENTED_EDGE('',*,*,#46728,.T.);
#62106=ORIENTED_EDGE('',*,*,#46708,.F.);
#62107=ORIENTED_EDGE('',*,*,#46729,.T.);
#62108=ORIENTED_EDGE('',*,*,#46710,.F.);
#62109=ORIENTED_EDGE('',*,*,#46730,.T.);
#62110=ORIENTED_EDGE('',*,*,#46731,.T.);
#62111=ORIENTED_EDGE('',*,*,#46732,.T.);
#62112=ORIENTED_EDGE('',*,*,#46733,.F.);
#62113=ORIENTED_EDGE('',*,*,#46734,.F.);
#62114=ORIENTED_EDGE('',*,*,#46735,.F.);
#62115=ORIENTED_EDGE('',*,*,#46736,.T.);
#62116=ORIENTED_EDGE('',*,*,#46734,.T.);
#62117=ORIENTED_EDGE('',*,*,#46737,.T.);
#62118=ORIENTED_EDGE('',*,*,#46738,.T.);
#62119=ORIENTED_EDGE('',*,*,#46739,.T.);
#62120=ORIENTED_EDGE('',*,*,#46740,.T.);
#62121=ORIENTED_EDGE('',*,*,#46741,.T.);
#62122=ORIENTED_EDGE('',*,*,#46742,.T.);
#62123=ORIENTED_EDGE('',*,*,#46743,.T.);
#62124=ORIENTED_EDGE('',*,*,#46744,.T.);
#62125=ORIENTED_EDGE('',*,*,#46745,.T.);
#62126=ORIENTED_EDGE('',*,*,#46746,.F.);
#62127=ORIENTED_EDGE('',*,*,#46747,.F.);
#62128=ORIENTED_EDGE('',*,*,#46748,.F.);
#62129=ORIENTED_EDGE('',*,*,#46749,.T.);
#62130=ORIENTED_EDGE('',*,*,#46747,.T.);
#62131=ORIENTED_EDGE('',*,*,#46750,.T.);
#62132=ORIENTED_EDGE('',*,*,#46751,.T.);
#62133=ORIENTED_EDGE('',*,*,#46752,.T.);
#62134=ORIENTED_EDGE('',*,*,#46478,.F.);
#62135=ORIENTED_EDGE('',*,*,#46753,.T.);
#62136=ORIENTED_EDGE('',*,*,#46731,.F.);
#62137=ORIENTED_EDGE('',*,*,#46754,.T.);
#62138=ORIENTED_EDGE('',*,*,#46751,.F.);
#62139=ORIENTED_EDGE('',*,*,#46755,.T.);
#62140=ORIENTED_EDGE('',*,*,#46255,.F.);
#62141=ORIENTED_EDGE('',*,*,#46756,.T.);
#62142=ORIENTED_EDGE('',*,*,#46742,.F.);
#62143=ORIENTED_EDGE('',*,*,#46757,.T.);
#62144=ORIENTED_EDGE('',*,*,#46744,.F.);
#62145=ORIENTED_EDGE('',*,*,#46758,.T.);
#62146=ORIENTED_EDGE('',*,*,#46738,.F.);
#62147=ORIENTED_EDGE('',*,*,#46759,.T.);
#62148=ORIENTED_EDGE('',*,*,#46740,.F.);
#62149=ORIENTED_EDGE('',*,*,#46760,.T.);
#62150=ORIENTED_EDGE('',*,*,#46761,.T.);
#62151=ORIENTED_EDGE('',*,*,#46762,.T.);
#62152=ORIENTED_EDGE('',*,*,#46763,.F.);
#62153=ORIENTED_EDGE('',*,*,#46764,.F.);
#62154=ORIENTED_EDGE('',*,*,#46765,.F.);
#62155=ORIENTED_EDGE('',*,*,#46766,.T.);
#62156=ORIENTED_EDGE('',*,*,#46764,.T.);
#62157=ORIENTED_EDGE('',*,*,#46767,.T.);
#62158=ORIENTED_EDGE('',*,*,#46768,.T.);
#62159=ORIENTED_EDGE('',*,*,#46769,.T.);
#62160=ORIENTED_EDGE('',*,*,#46770,.T.);
#62161=ORIENTED_EDGE('',*,*,#46771,.T.);
#62162=ORIENTED_EDGE('',*,*,#46772,.T.);
#62163=ORIENTED_EDGE('',*,*,#46773,.T.);
#62164=ORIENTED_EDGE('',*,*,#46774,.T.);
#62165=ORIENTED_EDGE('',*,*,#46775,.T.);
#62166=ORIENTED_EDGE('',*,*,#46776,.F.);
#62167=ORIENTED_EDGE('',*,*,#46777,.F.);
#62168=ORIENTED_EDGE('',*,*,#46778,.F.);
#62169=ORIENTED_EDGE('',*,*,#46779,.T.);
#62170=ORIENTED_EDGE('',*,*,#46777,.T.);
#62171=ORIENTED_EDGE('',*,*,#46780,.T.);
#62172=ORIENTED_EDGE('',*,*,#46781,.T.);
#62173=ORIENTED_EDGE('',*,*,#46782,.T.);
#62174=ORIENTED_EDGE('',*,*,#46484,.F.);
#62175=ORIENTED_EDGE('',*,*,#46783,.T.);
#62176=ORIENTED_EDGE('',*,*,#46761,.F.);
#62177=ORIENTED_EDGE('',*,*,#46784,.T.);
#62178=ORIENTED_EDGE('',*,*,#46781,.F.);
#62179=ORIENTED_EDGE('',*,*,#46785,.T.);
#62180=ORIENTED_EDGE('',*,*,#46249,.F.);
#62181=ORIENTED_EDGE('',*,*,#46786,.T.);
#62182=ORIENTED_EDGE('',*,*,#46772,.F.);
#62183=ORIENTED_EDGE('',*,*,#46787,.T.);
#62184=ORIENTED_EDGE('',*,*,#46774,.F.);
#62185=ORIENTED_EDGE('',*,*,#46788,.T.);
#62186=ORIENTED_EDGE('',*,*,#46768,.F.);
#62187=ORIENTED_EDGE('',*,*,#46789,.T.);
#62188=ORIENTED_EDGE('',*,*,#46770,.F.);
#62189=ORIENTED_EDGE('',*,*,#46790,.T.);
#62190=ORIENTED_EDGE('',*,*,#46791,.T.);
#62191=ORIENTED_EDGE('',*,*,#46792,.T.);
#62192=ORIENTED_EDGE('',*,*,#46793,.F.);
#62193=ORIENTED_EDGE('',*,*,#46794,.F.);
#62194=ORIENTED_EDGE('',*,*,#46795,.F.);
#62195=ORIENTED_EDGE('',*,*,#46796,.T.);
#62196=ORIENTED_EDGE('',*,*,#46794,.T.);
#62197=ORIENTED_EDGE('',*,*,#46797,.T.);
#62198=ORIENTED_EDGE('',*,*,#46798,.T.);
#62199=ORIENTED_EDGE('',*,*,#46799,.T.);
#62200=ORIENTED_EDGE('',*,*,#46800,.T.);
#62201=ORIENTED_EDGE('',*,*,#46801,.T.);
#62202=ORIENTED_EDGE('',*,*,#46802,.T.);
#62203=ORIENTED_EDGE('',*,*,#46803,.T.);
#62204=ORIENTED_EDGE('',*,*,#46804,.T.);
#62205=ORIENTED_EDGE('',*,*,#46805,.T.);
#62206=ORIENTED_EDGE('',*,*,#46806,.F.);
#62207=ORIENTED_EDGE('',*,*,#46807,.F.);
#62208=ORIENTED_EDGE('',*,*,#46808,.F.);
#62209=ORIENTED_EDGE('',*,*,#46809,.T.);
#62210=ORIENTED_EDGE('',*,*,#46807,.T.);
#62211=ORIENTED_EDGE('',*,*,#46810,.T.);
#62212=ORIENTED_EDGE('',*,*,#46811,.T.);
#62213=ORIENTED_EDGE('',*,*,#46812,.T.);
#62214=ORIENTED_EDGE('',*,*,#46490,.F.);
#62215=ORIENTED_EDGE('',*,*,#46813,.T.);
#62216=ORIENTED_EDGE('',*,*,#46791,.F.);
#62217=ORIENTED_EDGE('',*,*,#46814,.T.);
#62218=ORIENTED_EDGE('',*,*,#46811,.F.);
#62219=ORIENTED_EDGE('',*,*,#46815,.T.);
#62220=ORIENTED_EDGE('',*,*,#46243,.F.);
#62221=ORIENTED_EDGE('',*,*,#46816,.T.);
#62222=ORIENTED_EDGE('',*,*,#46802,.F.);
#62223=ORIENTED_EDGE('',*,*,#46817,.T.);
#62224=ORIENTED_EDGE('',*,*,#46804,.F.);
#62225=ORIENTED_EDGE('',*,*,#46818,.T.);
#62226=ORIENTED_EDGE('',*,*,#46798,.F.);
#62227=ORIENTED_EDGE('',*,*,#46819,.T.);
#62228=ORIENTED_EDGE('',*,*,#46800,.F.);
#62229=ORIENTED_EDGE('',*,*,#46820,.T.);
#62230=ORIENTED_EDGE('',*,*,#46821,.T.);
#62231=ORIENTED_EDGE('',*,*,#46822,.T.);
#62232=ORIENTED_EDGE('',*,*,#46823,.F.);
#62233=ORIENTED_EDGE('',*,*,#46824,.F.);
#62234=ORIENTED_EDGE('',*,*,#46825,.F.);
#62235=ORIENTED_EDGE('',*,*,#46826,.T.);
#62236=ORIENTED_EDGE('',*,*,#46824,.T.);
#62237=ORIENTED_EDGE('',*,*,#46827,.T.);
#62238=ORIENTED_EDGE('',*,*,#46828,.T.);
#62239=ORIENTED_EDGE('',*,*,#46829,.T.);
#62240=ORIENTED_EDGE('',*,*,#46830,.T.);
#62241=ORIENTED_EDGE('',*,*,#46831,.T.);
#62242=ORIENTED_EDGE('',*,*,#46832,.T.);
#62243=ORIENTED_EDGE('',*,*,#46833,.T.);
#62244=ORIENTED_EDGE('',*,*,#46834,.T.);
#62245=ORIENTED_EDGE('',*,*,#46835,.T.);
#62246=ORIENTED_EDGE('',*,*,#46836,.F.);
#62247=ORIENTED_EDGE('',*,*,#46837,.F.);
#62248=ORIENTED_EDGE('',*,*,#46838,.F.);
#62249=ORIENTED_EDGE('',*,*,#46839,.T.);
#62250=ORIENTED_EDGE('',*,*,#46837,.T.);
#62251=ORIENTED_EDGE('',*,*,#46840,.T.);
#62252=ORIENTED_EDGE('',*,*,#46841,.T.);
#62253=ORIENTED_EDGE('',*,*,#46842,.T.);
#62254=ORIENTED_EDGE('',*,*,#46496,.F.);
#62255=ORIENTED_EDGE('',*,*,#46843,.T.);
#62256=ORIENTED_EDGE('',*,*,#46821,.F.);
#62257=ORIENTED_EDGE('',*,*,#46844,.T.);
#62258=ORIENTED_EDGE('',*,*,#46841,.F.);
#62259=ORIENTED_EDGE('',*,*,#46845,.T.);
#62260=ORIENTED_EDGE('',*,*,#46237,.F.);
#62261=ORIENTED_EDGE('',*,*,#46846,.T.);
#62262=ORIENTED_EDGE('',*,*,#46832,.F.);
#62263=ORIENTED_EDGE('',*,*,#46847,.T.);
#62264=ORIENTED_EDGE('',*,*,#46834,.F.);
#62265=ORIENTED_EDGE('',*,*,#46848,.T.);
#62266=ORIENTED_EDGE('',*,*,#46828,.F.);
#62267=ORIENTED_EDGE('',*,*,#46849,.T.);
#62268=ORIENTED_EDGE('',*,*,#46830,.F.);
#62269=ORIENTED_EDGE('',*,*,#46850,.T.);
#62270=ORIENTED_EDGE('',*,*,#46851,.T.);
#62271=ORIENTED_EDGE('',*,*,#46852,.T.);
#62272=ORIENTED_EDGE('',*,*,#46853,.F.);
#62273=ORIENTED_EDGE('',*,*,#46854,.F.);
#62274=ORIENTED_EDGE('',*,*,#46855,.F.);
#62275=ORIENTED_EDGE('',*,*,#46856,.T.);
#62276=ORIENTED_EDGE('',*,*,#46854,.T.);
#62277=ORIENTED_EDGE('',*,*,#46857,.T.);
#62278=ORIENTED_EDGE('',*,*,#46858,.T.);
#62279=ORIENTED_EDGE('',*,*,#46859,.T.);
#62280=ORIENTED_EDGE('',*,*,#46860,.T.);
#62281=ORIENTED_EDGE('',*,*,#46861,.T.);
#62282=ORIENTED_EDGE('',*,*,#46862,.T.);
#62283=ORIENTED_EDGE('',*,*,#46863,.T.);
#62284=ORIENTED_EDGE('',*,*,#46864,.T.);
#62285=ORIENTED_EDGE('',*,*,#46865,.T.);
#62286=ORIENTED_EDGE('',*,*,#46866,.F.);
#62287=ORIENTED_EDGE('',*,*,#46867,.F.);
#62288=ORIENTED_EDGE('',*,*,#46868,.F.);
#62289=ORIENTED_EDGE('',*,*,#46869,.T.);
#62290=ORIENTED_EDGE('',*,*,#46867,.T.);
#62291=ORIENTED_EDGE('',*,*,#46870,.T.);
#62292=ORIENTED_EDGE('',*,*,#46871,.T.);
#62293=ORIENTED_EDGE('',*,*,#46872,.T.);
#62294=ORIENTED_EDGE('',*,*,#46502,.F.);
#62295=ORIENTED_EDGE('',*,*,#46873,.T.);
#62296=ORIENTED_EDGE('',*,*,#46851,.F.);
#62297=ORIENTED_EDGE('',*,*,#46874,.T.);
#62298=ORIENTED_EDGE('',*,*,#46871,.F.);
#62299=ORIENTED_EDGE('',*,*,#46875,.T.);
#62300=ORIENTED_EDGE('',*,*,#46231,.F.);
#62301=ORIENTED_EDGE('',*,*,#46876,.T.);
#62302=ORIENTED_EDGE('',*,*,#46862,.F.);
#62303=ORIENTED_EDGE('',*,*,#46877,.T.);
#62304=ORIENTED_EDGE('',*,*,#46864,.F.);
#62305=ORIENTED_EDGE('',*,*,#46878,.T.);
#62306=ORIENTED_EDGE('',*,*,#46858,.F.);
#62307=ORIENTED_EDGE('',*,*,#46879,.T.);
#62308=ORIENTED_EDGE('',*,*,#46860,.F.);
#62309=ORIENTED_EDGE('',*,*,#46880,.T.);
#62310=ORIENTED_EDGE('',*,*,#46881,.T.);
#62311=ORIENTED_EDGE('',*,*,#46882,.T.);
#62312=ORIENTED_EDGE('',*,*,#46883,.F.);
#62313=ORIENTED_EDGE('',*,*,#46884,.F.);
#62314=ORIENTED_EDGE('',*,*,#46885,.F.);
#62315=ORIENTED_EDGE('',*,*,#46886,.T.);
#62316=ORIENTED_EDGE('',*,*,#46884,.T.);
#62317=ORIENTED_EDGE('',*,*,#46887,.T.);
#62318=ORIENTED_EDGE('',*,*,#46888,.T.);
#62319=ORIENTED_EDGE('',*,*,#46889,.T.);
#62320=ORIENTED_EDGE('',*,*,#46890,.T.);
#62321=ORIENTED_EDGE('',*,*,#46891,.T.);
#62322=ORIENTED_EDGE('',*,*,#46892,.T.);
#62323=ORIENTED_EDGE('',*,*,#46893,.T.);
#62324=ORIENTED_EDGE('',*,*,#46894,.T.);
#62325=ORIENTED_EDGE('',*,*,#46895,.T.);
#62326=ORIENTED_EDGE('',*,*,#46896,.F.);
#62327=ORIENTED_EDGE('',*,*,#46897,.F.);
#62328=ORIENTED_EDGE('',*,*,#46898,.F.);
#62329=ORIENTED_EDGE('',*,*,#46899,.T.);
#62330=ORIENTED_EDGE('',*,*,#46897,.T.);
#62331=ORIENTED_EDGE('',*,*,#46900,.T.);
#62332=ORIENTED_EDGE('',*,*,#46901,.T.);
#62333=ORIENTED_EDGE('',*,*,#46902,.T.);
#62334=ORIENTED_EDGE('',*,*,#46508,.F.);
#62335=ORIENTED_EDGE('',*,*,#46903,.T.);
#62336=ORIENTED_EDGE('',*,*,#46881,.F.);
#62337=ORIENTED_EDGE('',*,*,#46904,.T.);
#62338=ORIENTED_EDGE('',*,*,#46901,.F.);
#62339=ORIENTED_EDGE('',*,*,#46905,.T.);
#62340=ORIENTED_EDGE('',*,*,#46225,.F.);
#62341=ORIENTED_EDGE('',*,*,#46906,.T.);
#62342=ORIENTED_EDGE('',*,*,#46892,.F.);
#62343=ORIENTED_EDGE('',*,*,#46907,.T.);
#62344=ORIENTED_EDGE('',*,*,#46894,.F.);
#62345=ORIENTED_EDGE('',*,*,#46908,.T.);
#62346=ORIENTED_EDGE('',*,*,#46888,.F.);
#62347=ORIENTED_EDGE('',*,*,#46909,.T.);
#62348=ORIENTED_EDGE('',*,*,#46890,.F.);
#62349=ORIENTED_EDGE('',*,*,#46910,.T.);
#62350=ORIENTED_EDGE('',*,*,#46911,.T.);
#62351=ORIENTED_EDGE('',*,*,#46912,.T.);
#62352=ORIENTED_EDGE('',*,*,#46913,.F.);
#62353=ORIENTED_EDGE('',*,*,#46914,.F.);
#62354=ORIENTED_EDGE('',*,*,#46915,.F.);
#62355=ORIENTED_EDGE('',*,*,#46916,.T.);
#62356=ORIENTED_EDGE('',*,*,#46914,.T.);
#62357=ORIENTED_EDGE('',*,*,#46917,.T.);
#62358=ORIENTED_EDGE('',*,*,#46918,.T.);
#62359=ORIENTED_EDGE('',*,*,#46919,.T.);
#62360=ORIENTED_EDGE('',*,*,#46920,.T.);
#62361=ORIENTED_EDGE('',*,*,#46921,.T.);
#62362=ORIENTED_EDGE('',*,*,#46922,.T.);
#62363=ORIENTED_EDGE('',*,*,#46923,.T.);
#62364=ORIENTED_EDGE('',*,*,#46924,.T.);
#62365=ORIENTED_EDGE('',*,*,#46925,.T.);
#62366=ORIENTED_EDGE('',*,*,#46926,.F.);
#62367=ORIENTED_EDGE('',*,*,#46927,.F.);
#62368=ORIENTED_EDGE('',*,*,#46928,.F.);
#62369=ORIENTED_EDGE('',*,*,#46929,.T.);
#62370=ORIENTED_EDGE('',*,*,#46927,.T.);
#62371=ORIENTED_EDGE('',*,*,#46930,.T.);
#62372=ORIENTED_EDGE('',*,*,#46931,.T.);
#62373=ORIENTED_EDGE('',*,*,#46932,.T.);
#62374=ORIENTED_EDGE('',*,*,#46514,.F.);
#62375=ORIENTED_EDGE('',*,*,#46933,.T.);
#62376=ORIENTED_EDGE('',*,*,#46911,.F.);
#62377=ORIENTED_EDGE('',*,*,#46934,.T.);
#62378=ORIENTED_EDGE('',*,*,#46931,.F.);
#62379=ORIENTED_EDGE('',*,*,#46935,.T.);
#62380=ORIENTED_EDGE('',*,*,#46219,.F.);
#62381=ORIENTED_EDGE('',*,*,#46936,.T.);
#62382=ORIENTED_EDGE('',*,*,#46922,.F.);
#62383=ORIENTED_EDGE('',*,*,#46937,.T.);
#62384=ORIENTED_EDGE('',*,*,#46924,.F.);
#62385=ORIENTED_EDGE('',*,*,#46938,.T.);
#62386=ORIENTED_EDGE('',*,*,#46918,.F.);
#62387=ORIENTED_EDGE('',*,*,#46939,.T.);
#62388=ORIENTED_EDGE('',*,*,#46920,.F.);
#62389=ORIENTED_EDGE('',*,*,#46940,.T.);
#62390=ORIENTED_EDGE('',*,*,#46941,.T.);
#62391=ORIENTED_EDGE('',*,*,#46942,.T.);
#62392=ORIENTED_EDGE('',*,*,#46943,.F.);
#62393=ORIENTED_EDGE('',*,*,#46944,.F.);
#62394=ORIENTED_EDGE('',*,*,#46945,.F.);
#62395=ORIENTED_EDGE('',*,*,#46946,.T.);
#62396=ORIENTED_EDGE('',*,*,#46944,.T.);
#62397=ORIENTED_EDGE('',*,*,#46947,.T.);
#62398=ORIENTED_EDGE('',*,*,#46948,.T.);
#62399=ORIENTED_EDGE('',*,*,#46949,.T.);
#62400=ORIENTED_EDGE('',*,*,#46950,.T.);
#62401=ORIENTED_EDGE('',*,*,#46951,.T.);
#62402=ORIENTED_EDGE('',*,*,#46952,.T.);
#62403=ORIENTED_EDGE('',*,*,#46953,.T.);
#62404=ORIENTED_EDGE('',*,*,#46954,.T.);
#62405=ORIENTED_EDGE('',*,*,#46955,.T.);
#62406=ORIENTED_EDGE('',*,*,#46956,.F.);
#62407=ORIENTED_EDGE('',*,*,#46957,.F.);
#62408=ORIENTED_EDGE('',*,*,#46958,.F.);
#62409=ORIENTED_EDGE('',*,*,#46959,.T.);
#62410=ORIENTED_EDGE('',*,*,#46957,.T.);
#62411=ORIENTED_EDGE('',*,*,#46960,.T.);
#62412=ORIENTED_EDGE('',*,*,#46961,.T.);
#62413=ORIENTED_EDGE('',*,*,#46962,.T.);
#62414=ORIENTED_EDGE('',*,*,#46520,.F.);
#62415=ORIENTED_EDGE('',*,*,#46963,.T.);
#62416=ORIENTED_EDGE('',*,*,#46941,.F.);
#62417=ORIENTED_EDGE('',*,*,#46964,.T.);
#62418=ORIENTED_EDGE('',*,*,#46961,.F.);
#62419=ORIENTED_EDGE('',*,*,#46965,.T.);
#62420=ORIENTED_EDGE('',*,*,#46213,.F.);
#62421=ORIENTED_EDGE('',*,*,#46966,.T.);
#62422=ORIENTED_EDGE('',*,*,#46952,.F.);
#62423=ORIENTED_EDGE('',*,*,#46967,.T.);
#62424=ORIENTED_EDGE('',*,*,#46954,.F.);
#62425=ORIENTED_EDGE('',*,*,#46968,.T.);
#62426=ORIENTED_EDGE('',*,*,#46948,.F.);
#62427=ORIENTED_EDGE('',*,*,#46969,.T.);
#62428=ORIENTED_EDGE('',*,*,#46950,.F.);
#62429=ORIENTED_EDGE('',*,*,#46970,.T.);
#62430=ORIENTED_EDGE('',*,*,#46971,.T.);
#62431=ORIENTED_EDGE('',*,*,#46972,.T.);
#62432=ORIENTED_EDGE('',*,*,#46973,.F.);
#62433=ORIENTED_EDGE('',*,*,#46974,.F.);
#62434=ORIENTED_EDGE('',*,*,#46975,.F.);
#62435=ORIENTED_EDGE('',*,*,#46976,.T.);
#62436=ORIENTED_EDGE('',*,*,#46974,.T.);
#62437=ORIENTED_EDGE('',*,*,#46977,.T.);
#62438=ORIENTED_EDGE('',*,*,#46978,.T.);
#62439=ORIENTED_EDGE('',*,*,#46979,.T.);
#62440=ORIENTED_EDGE('',*,*,#46980,.T.);
#62441=ORIENTED_EDGE('',*,*,#46981,.T.);
#62442=ORIENTED_EDGE('',*,*,#46982,.T.);
#62443=ORIENTED_EDGE('',*,*,#46983,.T.);
#62444=ORIENTED_EDGE('',*,*,#46984,.T.);
#62445=ORIENTED_EDGE('',*,*,#46985,.T.);
#62446=ORIENTED_EDGE('',*,*,#46986,.F.);
#62447=ORIENTED_EDGE('',*,*,#46987,.F.);
#62448=ORIENTED_EDGE('',*,*,#46988,.F.);
#62449=ORIENTED_EDGE('',*,*,#46989,.T.);
#62450=ORIENTED_EDGE('',*,*,#46987,.T.);
#62451=ORIENTED_EDGE('',*,*,#46990,.T.);
#62452=ORIENTED_EDGE('',*,*,#46991,.T.);
#62453=ORIENTED_EDGE('',*,*,#46992,.T.);
#62454=ORIENTED_EDGE('',*,*,#46526,.F.);
#62455=ORIENTED_EDGE('',*,*,#46993,.T.);
#62456=ORIENTED_EDGE('',*,*,#46971,.F.);
#62457=ORIENTED_EDGE('',*,*,#46994,.T.);
#62458=ORIENTED_EDGE('',*,*,#46991,.F.);
#62459=ORIENTED_EDGE('',*,*,#46995,.T.);
#62460=ORIENTED_EDGE('',*,*,#46207,.F.);
#62461=ORIENTED_EDGE('',*,*,#46996,.T.);
#62462=ORIENTED_EDGE('',*,*,#46982,.F.);
#62463=ORIENTED_EDGE('',*,*,#46997,.T.);
#62464=ORIENTED_EDGE('',*,*,#46984,.F.);
#62465=ORIENTED_EDGE('',*,*,#46998,.T.);
#62466=ORIENTED_EDGE('',*,*,#46978,.F.);
#62467=ORIENTED_EDGE('',*,*,#46999,.T.);
#62468=ORIENTED_EDGE('',*,*,#46980,.F.);
#62469=ORIENTED_EDGE('',*,*,#47000,.T.);
#62470=ORIENTED_EDGE('',*,*,#47001,.T.);
#62471=ORIENTED_EDGE('',*,*,#47002,.T.);
#62472=ORIENTED_EDGE('',*,*,#47003,.F.);
#62473=ORIENTED_EDGE('',*,*,#47004,.F.);
#62474=ORIENTED_EDGE('',*,*,#47005,.F.);
#62475=ORIENTED_EDGE('',*,*,#47006,.T.);
#62476=ORIENTED_EDGE('',*,*,#47004,.T.);
#62477=ORIENTED_EDGE('',*,*,#47007,.T.);
#62478=ORIENTED_EDGE('',*,*,#47008,.T.);
#62479=ORIENTED_EDGE('',*,*,#47009,.T.);
#62480=ORIENTED_EDGE('',*,*,#47010,.T.);
#62481=ORIENTED_EDGE('',*,*,#47011,.T.);
#62482=ORIENTED_EDGE('',*,*,#47012,.T.);
#62483=ORIENTED_EDGE('',*,*,#47013,.T.);
#62484=ORIENTED_EDGE('',*,*,#47014,.T.);
#62485=ORIENTED_EDGE('',*,*,#47015,.T.);
#62486=ORIENTED_EDGE('',*,*,#47016,.F.);
#62487=ORIENTED_EDGE('',*,*,#47017,.F.);
#62488=ORIENTED_EDGE('',*,*,#47018,.F.);
#62489=ORIENTED_EDGE('',*,*,#47019,.T.);
#62490=ORIENTED_EDGE('',*,*,#47017,.T.);
#62491=ORIENTED_EDGE('',*,*,#47020,.T.);
#62492=ORIENTED_EDGE('',*,*,#47021,.T.);
#62493=ORIENTED_EDGE('',*,*,#47022,.T.);
#62494=ORIENTED_EDGE('',*,*,#46532,.F.);
#62495=ORIENTED_EDGE('',*,*,#47023,.T.);
#62496=ORIENTED_EDGE('',*,*,#47001,.F.);
#62497=ORIENTED_EDGE('',*,*,#47024,.T.);
#62498=ORIENTED_EDGE('',*,*,#47021,.F.);
#62499=ORIENTED_EDGE('',*,*,#47025,.T.);
#62500=ORIENTED_EDGE('',*,*,#46201,.F.);
#62501=ORIENTED_EDGE('',*,*,#47026,.T.);
#62502=ORIENTED_EDGE('',*,*,#47012,.F.);
#62503=ORIENTED_EDGE('',*,*,#47027,.T.);
#62504=ORIENTED_EDGE('',*,*,#47014,.F.);
#62505=ORIENTED_EDGE('',*,*,#47028,.T.);
#62506=ORIENTED_EDGE('',*,*,#47008,.F.);
#62507=ORIENTED_EDGE('',*,*,#47029,.T.);
#62508=ORIENTED_EDGE('',*,*,#47010,.F.);
#62509=ORIENTED_EDGE('',*,*,#47030,.T.);
#62510=ORIENTED_EDGE('',*,*,#47031,.T.);
#62511=ORIENTED_EDGE('',*,*,#47032,.T.);
#62512=ORIENTED_EDGE('',*,*,#47033,.F.);
#62513=ORIENTED_EDGE('',*,*,#47034,.F.);
#62514=ORIENTED_EDGE('',*,*,#47035,.F.);
#62515=ORIENTED_EDGE('',*,*,#47036,.T.);
#62516=ORIENTED_EDGE('',*,*,#47034,.T.);
#62517=ORIENTED_EDGE('',*,*,#47037,.T.);
#62518=ORIENTED_EDGE('',*,*,#47038,.T.);
#62519=ORIENTED_EDGE('',*,*,#47039,.T.);
#62520=ORIENTED_EDGE('',*,*,#47040,.T.);
#62521=ORIENTED_EDGE('',*,*,#47041,.T.);
#62522=ORIENTED_EDGE('',*,*,#47042,.T.);
#62523=ORIENTED_EDGE('',*,*,#47043,.T.);
#62524=ORIENTED_EDGE('',*,*,#47044,.T.);
#62525=ORIENTED_EDGE('',*,*,#47045,.T.);
#62526=ORIENTED_EDGE('',*,*,#47046,.F.);
#62527=ORIENTED_EDGE('',*,*,#47047,.F.);
#62528=ORIENTED_EDGE('',*,*,#47048,.F.);
#62529=ORIENTED_EDGE('',*,*,#47049,.T.);
#62530=ORIENTED_EDGE('',*,*,#47047,.T.);
#62531=ORIENTED_EDGE('',*,*,#47050,.T.);
#62532=ORIENTED_EDGE('',*,*,#47051,.T.);
#62533=ORIENTED_EDGE('',*,*,#47052,.T.);
#62534=ORIENTED_EDGE('',*,*,#46538,.F.);
#62535=ORIENTED_EDGE('',*,*,#47053,.T.);
#62536=ORIENTED_EDGE('',*,*,#47031,.F.);
#62537=ORIENTED_EDGE('',*,*,#47054,.T.);
#62538=ORIENTED_EDGE('',*,*,#47051,.F.);
#62539=ORIENTED_EDGE('',*,*,#47055,.T.);
#62540=ORIENTED_EDGE('',*,*,#46195,.F.);
#62541=ORIENTED_EDGE('',*,*,#47056,.T.);
#62542=ORIENTED_EDGE('',*,*,#47042,.F.);
#62543=ORIENTED_EDGE('',*,*,#47057,.T.);
#62544=ORIENTED_EDGE('',*,*,#47044,.F.);
#62545=ORIENTED_EDGE('',*,*,#47058,.T.);
#62546=ORIENTED_EDGE('',*,*,#47038,.F.);
#62547=ORIENTED_EDGE('',*,*,#47059,.T.);
#62548=ORIENTED_EDGE('',*,*,#47040,.F.);
#62549=ORIENTED_EDGE('',*,*,#47060,.T.);
#62550=ORIENTED_EDGE('',*,*,#47061,.T.);
#62551=ORIENTED_EDGE('',*,*,#47062,.T.);
#62552=ORIENTED_EDGE('',*,*,#47063,.F.);
#62553=ORIENTED_EDGE('',*,*,#47064,.F.);
#62554=ORIENTED_EDGE('',*,*,#47065,.F.);
#62555=ORIENTED_EDGE('',*,*,#47066,.T.);
#62556=ORIENTED_EDGE('',*,*,#47064,.T.);
#62557=ORIENTED_EDGE('',*,*,#47067,.T.);
#62558=ORIENTED_EDGE('',*,*,#47068,.T.);
#62559=ORIENTED_EDGE('',*,*,#47069,.T.);
#62560=ORIENTED_EDGE('',*,*,#47070,.T.);
#62561=ORIENTED_EDGE('',*,*,#47071,.T.);
#62562=ORIENTED_EDGE('',*,*,#47072,.T.);
#62563=ORIENTED_EDGE('',*,*,#47073,.T.);
#62564=ORIENTED_EDGE('',*,*,#47074,.T.);
#62565=ORIENTED_EDGE('',*,*,#47075,.T.);
#62566=ORIENTED_EDGE('',*,*,#47076,.F.);
#62567=ORIENTED_EDGE('',*,*,#47077,.F.);
#62568=ORIENTED_EDGE('',*,*,#47078,.F.);
#62569=ORIENTED_EDGE('',*,*,#47079,.T.);
#62570=ORIENTED_EDGE('',*,*,#47077,.T.);
#62571=ORIENTED_EDGE('',*,*,#47080,.T.);
#62572=ORIENTED_EDGE('',*,*,#47081,.T.);
#62573=ORIENTED_EDGE('',*,*,#47082,.T.);
#62574=ORIENTED_EDGE('',*,*,#46544,.F.);
#62575=ORIENTED_EDGE('',*,*,#47083,.T.);
#62576=ORIENTED_EDGE('',*,*,#47061,.F.);
#62577=ORIENTED_EDGE('',*,*,#47084,.T.);
#62578=ORIENTED_EDGE('',*,*,#47081,.F.);
#62579=ORIENTED_EDGE('',*,*,#47085,.T.);
#62580=ORIENTED_EDGE('',*,*,#46189,.F.);
#62581=ORIENTED_EDGE('',*,*,#47086,.T.);
#62582=ORIENTED_EDGE('',*,*,#47072,.F.);
#62583=ORIENTED_EDGE('',*,*,#47087,.T.);
#62584=ORIENTED_EDGE('',*,*,#47074,.F.);
#62585=ORIENTED_EDGE('',*,*,#47088,.T.);
#62586=ORIENTED_EDGE('',*,*,#47068,.F.);
#62587=ORIENTED_EDGE('',*,*,#47089,.T.);
#62588=ORIENTED_EDGE('',*,*,#47070,.F.);
#62589=ORIENTED_EDGE('',*,*,#47090,.T.);
#62590=ORIENTED_EDGE('',*,*,#47091,.T.);
#62591=ORIENTED_EDGE('',*,*,#47092,.T.);
#62592=ORIENTED_EDGE('',*,*,#47093,.F.);
#62593=ORIENTED_EDGE('',*,*,#47094,.F.);
#62594=ORIENTED_EDGE('',*,*,#47095,.F.);
#62595=ORIENTED_EDGE('',*,*,#47096,.T.);
#62596=ORIENTED_EDGE('',*,*,#47094,.T.);
#62597=ORIENTED_EDGE('',*,*,#47097,.T.);
#62598=ORIENTED_EDGE('',*,*,#47098,.T.);
#62599=ORIENTED_EDGE('',*,*,#47099,.T.);
#62600=ORIENTED_EDGE('',*,*,#47100,.T.);
#62601=ORIENTED_EDGE('',*,*,#47101,.T.);
#62602=ORIENTED_EDGE('',*,*,#47102,.T.);
#62603=ORIENTED_EDGE('',*,*,#47103,.T.);
#62604=ORIENTED_EDGE('',*,*,#47104,.T.);
#62605=ORIENTED_EDGE('',*,*,#47105,.T.);
#62606=ORIENTED_EDGE('',*,*,#47106,.F.);
#62607=ORIENTED_EDGE('',*,*,#47107,.F.);
#62608=ORIENTED_EDGE('',*,*,#47108,.F.);
#62609=ORIENTED_EDGE('',*,*,#47109,.T.);
#62610=ORIENTED_EDGE('',*,*,#47107,.T.);
#62611=ORIENTED_EDGE('',*,*,#47110,.T.);
#62612=ORIENTED_EDGE('',*,*,#47111,.T.);
#62613=ORIENTED_EDGE('',*,*,#47112,.T.);
#62614=ORIENTED_EDGE('',*,*,#46549,.F.);
#62615=ORIENTED_EDGE('',*,*,#47113,.T.);
#62616=ORIENTED_EDGE('',*,*,#47091,.F.);
#62617=ORIENTED_EDGE('',*,*,#47114,.T.);
#62618=ORIENTED_EDGE('',*,*,#47111,.F.);
#62619=ORIENTED_EDGE('',*,*,#47115,.T.);
#62620=ORIENTED_EDGE('',*,*,#46184,.F.);
#62621=ORIENTED_EDGE('',*,*,#47116,.T.);
#62622=ORIENTED_EDGE('',*,*,#47102,.F.);
#62623=ORIENTED_EDGE('',*,*,#47117,.T.);
#62624=ORIENTED_EDGE('',*,*,#47104,.F.);
#62625=ORIENTED_EDGE('',*,*,#47118,.T.);
#62626=ORIENTED_EDGE('',*,*,#47098,.F.);
#62627=ORIENTED_EDGE('',*,*,#47119,.T.);
#62628=ORIENTED_EDGE('',*,*,#47100,.F.);
#62629=ORIENTED_EDGE('',*,*,#47120,.T.);
#62630=ORIENTED_EDGE('',*,*,#47121,.T.);
#62631=ORIENTED_EDGE('',*,*,#47122,.T.);
#62632=ORIENTED_EDGE('',*,*,#47123,.F.);
#62633=ORIENTED_EDGE('',*,*,#47124,.F.);
#62634=ORIENTED_EDGE('',*,*,#47125,.F.);
#62635=ORIENTED_EDGE('',*,*,#47126,.T.);
#62636=ORIENTED_EDGE('',*,*,#47124,.T.);
#62637=ORIENTED_EDGE('',*,*,#47127,.T.);
#62638=ORIENTED_EDGE('',*,*,#47128,.T.);
#62639=ORIENTED_EDGE('',*,*,#47129,.T.);
#62640=ORIENTED_EDGE('',*,*,#47130,.T.);
#62641=ORIENTED_EDGE('',*,*,#47131,.T.);
#62642=ORIENTED_EDGE('',*,*,#47132,.T.);
#62643=ORIENTED_EDGE('',*,*,#47133,.T.);
#62644=ORIENTED_EDGE('',*,*,#47134,.T.);
#62645=ORIENTED_EDGE('',*,*,#47135,.T.);
#62646=ORIENTED_EDGE('',*,*,#47136,.F.);
#62647=ORIENTED_EDGE('',*,*,#47137,.F.);
#62648=ORIENTED_EDGE('',*,*,#47138,.F.);
#62649=ORIENTED_EDGE('',*,*,#47139,.T.);
#62650=ORIENTED_EDGE('',*,*,#47137,.T.);
#62651=ORIENTED_EDGE('',*,*,#47140,.T.);
#62652=ORIENTED_EDGE('',*,*,#47141,.T.);
#62653=ORIENTED_EDGE('',*,*,#47142,.T.);
#62654=ORIENTED_EDGE('',*,*,#46555,.F.);
#62655=ORIENTED_EDGE('',*,*,#47143,.T.);
#62656=ORIENTED_EDGE('',*,*,#47121,.F.);
#62657=ORIENTED_EDGE('',*,*,#47144,.T.);
#62658=ORIENTED_EDGE('',*,*,#47141,.F.);
#62659=ORIENTED_EDGE('',*,*,#47145,.T.);
#62660=ORIENTED_EDGE('',*,*,#46178,.F.);
#62661=ORIENTED_EDGE('',*,*,#47146,.T.);
#62662=ORIENTED_EDGE('',*,*,#47132,.F.);
#62663=ORIENTED_EDGE('',*,*,#47147,.T.);
#62664=ORIENTED_EDGE('',*,*,#47134,.F.);
#62665=ORIENTED_EDGE('',*,*,#47148,.T.);
#62666=ORIENTED_EDGE('',*,*,#47128,.F.);
#62667=ORIENTED_EDGE('',*,*,#47149,.T.);
#62668=ORIENTED_EDGE('',*,*,#47130,.F.);
#62669=ORIENTED_EDGE('',*,*,#47150,.T.);
#62670=ORIENTED_EDGE('',*,*,#47151,.T.);
#62671=ORIENTED_EDGE('',*,*,#47152,.T.);
#62672=ORIENTED_EDGE('',*,*,#47153,.F.);
#62673=ORIENTED_EDGE('',*,*,#47154,.F.);
#62674=ORIENTED_EDGE('',*,*,#47155,.F.);
#62675=ORIENTED_EDGE('',*,*,#47156,.T.);
#62676=ORIENTED_EDGE('',*,*,#47154,.T.);
#62677=ORIENTED_EDGE('',*,*,#47157,.T.);
#62678=ORIENTED_EDGE('',*,*,#47158,.T.);
#62679=ORIENTED_EDGE('',*,*,#47159,.T.);
#62680=ORIENTED_EDGE('',*,*,#47160,.T.);
#62681=ORIENTED_EDGE('',*,*,#47161,.T.);
#62682=ORIENTED_EDGE('',*,*,#47162,.T.);
#62683=ORIENTED_EDGE('',*,*,#47163,.T.);
#62684=ORIENTED_EDGE('',*,*,#47164,.T.);
#62685=ORIENTED_EDGE('',*,*,#47165,.T.);
#62686=ORIENTED_EDGE('',*,*,#47166,.F.);
#62687=ORIENTED_EDGE('',*,*,#47167,.F.);
#62688=ORIENTED_EDGE('',*,*,#47168,.F.);
#62689=ORIENTED_EDGE('',*,*,#47169,.T.);
#62690=ORIENTED_EDGE('',*,*,#47167,.T.);
#62691=ORIENTED_EDGE('',*,*,#47170,.T.);
#62692=ORIENTED_EDGE('',*,*,#47171,.T.);
#62693=ORIENTED_EDGE('',*,*,#47172,.T.);
#62694=ORIENTED_EDGE('',*,*,#46561,.F.);
#62695=ORIENTED_EDGE('',*,*,#47173,.T.);
#62696=ORIENTED_EDGE('',*,*,#47151,.F.);
#62697=ORIENTED_EDGE('',*,*,#47174,.T.);
#62698=ORIENTED_EDGE('',*,*,#47171,.F.);
#62699=ORIENTED_EDGE('',*,*,#47175,.T.);
#62700=ORIENTED_EDGE('',*,*,#46172,.F.);
#62701=ORIENTED_EDGE('',*,*,#47176,.T.);
#62702=ORIENTED_EDGE('',*,*,#47162,.F.);
#62703=ORIENTED_EDGE('',*,*,#47177,.T.);
#62704=ORIENTED_EDGE('',*,*,#47164,.F.);
#62705=ORIENTED_EDGE('',*,*,#47178,.T.);
#62706=ORIENTED_EDGE('',*,*,#47158,.F.);
#62707=ORIENTED_EDGE('',*,*,#47179,.T.);
#62708=ORIENTED_EDGE('',*,*,#47160,.F.);
#62709=ORIENTED_EDGE('',*,*,#47180,.T.);
#62710=ORIENTED_EDGE('',*,*,#47181,.T.);
#62711=ORIENTED_EDGE('',*,*,#47182,.T.);
#62712=ORIENTED_EDGE('',*,*,#47183,.F.);
#62713=ORIENTED_EDGE('',*,*,#47184,.F.);
#62714=ORIENTED_EDGE('',*,*,#47185,.F.);
#62715=ORIENTED_EDGE('',*,*,#47186,.T.);
#62716=ORIENTED_EDGE('',*,*,#47184,.T.);
#62717=ORIENTED_EDGE('',*,*,#47187,.T.);
#62718=ORIENTED_EDGE('',*,*,#47188,.T.);
#62719=ORIENTED_EDGE('',*,*,#47189,.T.);
#62720=ORIENTED_EDGE('',*,*,#47190,.T.);
#62721=ORIENTED_EDGE('',*,*,#47191,.T.);
#62722=ORIENTED_EDGE('',*,*,#47192,.T.);
#62723=ORIENTED_EDGE('',*,*,#47193,.T.);
#62724=ORIENTED_EDGE('',*,*,#47194,.T.);
#62725=ORIENTED_EDGE('',*,*,#47195,.T.);
#62726=ORIENTED_EDGE('',*,*,#47196,.F.);
#62727=ORIENTED_EDGE('',*,*,#47197,.F.);
#62728=ORIENTED_EDGE('',*,*,#47198,.F.);
#62729=ORIENTED_EDGE('',*,*,#47199,.T.);
#62730=ORIENTED_EDGE('',*,*,#47197,.T.);
#62731=ORIENTED_EDGE('',*,*,#47200,.T.);
#62732=ORIENTED_EDGE('',*,*,#47201,.T.);
#62733=ORIENTED_EDGE('',*,*,#47202,.T.);
#62734=ORIENTED_EDGE('',*,*,#46567,.F.);
#62735=ORIENTED_EDGE('',*,*,#47203,.T.);
#62736=ORIENTED_EDGE('',*,*,#47181,.F.);
#62737=ORIENTED_EDGE('',*,*,#47204,.T.);
#62738=ORIENTED_EDGE('',*,*,#47201,.F.);
#62739=ORIENTED_EDGE('',*,*,#47205,.T.);
#62740=ORIENTED_EDGE('',*,*,#46166,.F.);
#62741=ORIENTED_EDGE('',*,*,#47206,.T.);
#62742=ORIENTED_EDGE('',*,*,#47192,.F.);
#62743=ORIENTED_EDGE('',*,*,#47207,.T.);
#62744=ORIENTED_EDGE('',*,*,#47194,.F.);
#62745=ORIENTED_EDGE('',*,*,#47208,.T.);
#62746=ORIENTED_EDGE('',*,*,#47188,.F.);
#62747=ORIENTED_EDGE('',*,*,#47209,.T.);
#62748=ORIENTED_EDGE('',*,*,#47190,.F.);
#62749=ORIENTED_EDGE('',*,*,#47210,.T.);
#62750=ORIENTED_EDGE('',*,*,#47211,.T.);
#62751=ORIENTED_EDGE('',*,*,#47212,.T.);
#62752=ORIENTED_EDGE('',*,*,#47213,.F.);
#62753=ORIENTED_EDGE('',*,*,#47214,.F.);
#62754=ORIENTED_EDGE('',*,*,#47215,.F.);
#62755=ORIENTED_EDGE('',*,*,#47216,.T.);
#62756=ORIENTED_EDGE('',*,*,#47214,.T.);
#62757=ORIENTED_EDGE('',*,*,#47217,.T.);
#62758=ORIENTED_EDGE('',*,*,#47218,.T.);
#62759=ORIENTED_EDGE('',*,*,#47219,.T.);
#62760=ORIENTED_EDGE('',*,*,#47220,.T.);
#62761=ORIENTED_EDGE('',*,*,#47221,.T.);
#62762=ORIENTED_EDGE('',*,*,#47222,.T.);
#62763=ORIENTED_EDGE('',*,*,#47223,.T.);
#62764=ORIENTED_EDGE('',*,*,#47224,.T.);
#62765=ORIENTED_EDGE('',*,*,#47225,.T.);
#62766=ORIENTED_EDGE('',*,*,#47226,.F.);
#62767=ORIENTED_EDGE('',*,*,#47227,.F.);
#62768=ORIENTED_EDGE('',*,*,#47228,.F.);
#62769=ORIENTED_EDGE('',*,*,#47229,.T.);
#62770=ORIENTED_EDGE('',*,*,#47227,.T.);
#62771=ORIENTED_EDGE('',*,*,#47230,.T.);
#62772=ORIENTED_EDGE('',*,*,#47231,.T.);
#62773=ORIENTED_EDGE('',*,*,#47232,.T.);
#62774=ORIENTED_EDGE('',*,*,#46573,.F.);
#62775=ORIENTED_EDGE('',*,*,#47233,.T.);
#62776=ORIENTED_EDGE('',*,*,#47211,.F.);
#62777=ORIENTED_EDGE('',*,*,#47234,.T.);
#62778=ORIENTED_EDGE('',*,*,#47231,.F.);
#62779=ORIENTED_EDGE('',*,*,#47235,.T.);
#62780=ORIENTED_EDGE('',*,*,#46160,.F.);
#62781=ORIENTED_EDGE('',*,*,#47236,.T.);
#62782=ORIENTED_EDGE('',*,*,#47222,.F.);
#62783=ORIENTED_EDGE('',*,*,#47237,.T.);
#62784=ORIENTED_EDGE('',*,*,#47224,.F.);
#62785=ORIENTED_EDGE('',*,*,#47238,.T.);
#62786=ORIENTED_EDGE('',*,*,#47218,.F.);
#62787=ORIENTED_EDGE('',*,*,#47239,.T.);
#62788=ORIENTED_EDGE('',*,*,#47220,.F.);
#62789=ORIENTED_EDGE('',*,*,#47240,.T.);
#62790=ORIENTED_EDGE('',*,*,#47241,.T.);
#62791=ORIENTED_EDGE('',*,*,#47242,.T.);
#62792=ORIENTED_EDGE('',*,*,#47243,.F.);
#62793=ORIENTED_EDGE('',*,*,#47244,.F.);
#62794=ORIENTED_EDGE('',*,*,#47245,.F.);
#62795=ORIENTED_EDGE('',*,*,#47246,.T.);
#62796=ORIENTED_EDGE('',*,*,#47244,.T.);
#62797=ORIENTED_EDGE('',*,*,#47247,.T.);
#62798=ORIENTED_EDGE('',*,*,#47248,.T.);
#62799=ORIENTED_EDGE('',*,*,#47249,.T.);
#62800=ORIENTED_EDGE('',*,*,#47250,.T.);
#62801=ORIENTED_EDGE('',*,*,#47251,.T.);
#62802=ORIENTED_EDGE('',*,*,#47252,.T.);
#62803=ORIENTED_EDGE('',*,*,#47253,.T.);
#62804=ORIENTED_EDGE('',*,*,#47254,.T.);
#62805=ORIENTED_EDGE('',*,*,#47255,.T.);
#62806=ORIENTED_EDGE('',*,*,#47256,.F.);
#62807=ORIENTED_EDGE('',*,*,#47257,.F.);
#62808=ORIENTED_EDGE('',*,*,#47258,.F.);
#62809=ORIENTED_EDGE('',*,*,#47259,.T.);
#62810=ORIENTED_EDGE('',*,*,#47257,.T.);
#62811=ORIENTED_EDGE('',*,*,#47260,.T.);
#62812=ORIENTED_EDGE('',*,*,#47261,.T.);
#62813=ORIENTED_EDGE('',*,*,#47262,.T.);
#62814=ORIENTED_EDGE('',*,*,#46579,.F.);
#62815=ORIENTED_EDGE('',*,*,#47263,.T.);
#62816=ORIENTED_EDGE('',*,*,#47241,.F.);
#62817=ORIENTED_EDGE('',*,*,#47264,.T.);
#62818=ORIENTED_EDGE('',*,*,#47261,.F.);
#62819=ORIENTED_EDGE('',*,*,#47265,.T.);
#62820=ORIENTED_EDGE('',*,*,#46154,.F.);
#62821=ORIENTED_EDGE('',*,*,#47266,.T.);
#62822=ORIENTED_EDGE('',*,*,#47252,.F.);
#62823=ORIENTED_EDGE('',*,*,#47267,.T.);
#62824=ORIENTED_EDGE('',*,*,#47254,.F.);
#62825=ORIENTED_EDGE('',*,*,#47268,.T.);
#62826=ORIENTED_EDGE('',*,*,#47248,.F.);
#62827=ORIENTED_EDGE('',*,*,#47269,.T.);
#62828=ORIENTED_EDGE('',*,*,#47250,.F.);
#62829=ORIENTED_EDGE('',*,*,#47270,.T.);
#62830=ORIENTED_EDGE('',*,*,#47271,.T.);
#62831=ORIENTED_EDGE('',*,*,#47272,.T.);
#62832=ORIENTED_EDGE('',*,*,#47273,.F.);
#62833=ORIENTED_EDGE('',*,*,#47274,.F.);
#62834=ORIENTED_EDGE('',*,*,#47275,.F.);
#62835=ORIENTED_EDGE('',*,*,#47276,.T.);
#62836=ORIENTED_EDGE('',*,*,#47274,.T.);
#62837=ORIENTED_EDGE('',*,*,#47277,.T.);
#62838=ORIENTED_EDGE('',*,*,#47278,.T.);
#62839=ORIENTED_EDGE('',*,*,#47279,.T.);
#62840=ORIENTED_EDGE('',*,*,#47280,.T.);
#62841=ORIENTED_EDGE('',*,*,#47281,.T.);
#62842=ORIENTED_EDGE('',*,*,#47282,.T.);
#62843=ORIENTED_EDGE('',*,*,#47283,.T.);
#62844=ORIENTED_EDGE('',*,*,#47284,.T.);
#62845=ORIENTED_EDGE('',*,*,#47285,.T.);
#62846=ORIENTED_EDGE('',*,*,#47286,.F.);
#62847=ORIENTED_EDGE('',*,*,#47287,.F.);
#62848=ORIENTED_EDGE('',*,*,#47288,.F.);
#62849=ORIENTED_EDGE('',*,*,#47289,.T.);
#62850=ORIENTED_EDGE('',*,*,#47287,.T.);
#62851=ORIENTED_EDGE('',*,*,#47290,.T.);
#62852=ORIENTED_EDGE('',*,*,#47291,.T.);
#62853=ORIENTED_EDGE('',*,*,#47292,.T.);
#62854=ORIENTED_EDGE('',*,*,#46585,.F.);
#62855=ORIENTED_EDGE('',*,*,#47293,.T.);
#62856=ORIENTED_EDGE('',*,*,#47271,.F.);
#62857=ORIENTED_EDGE('',*,*,#47294,.T.);
#62858=ORIENTED_EDGE('',*,*,#47291,.F.);
#62859=ORIENTED_EDGE('',*,*,#47295,.T.);
#62860=ORIENTED_EDGE('',*,*,#46148,.F.);
#62861=ORIENTED_EDGE('',*,*,#47296,.T.);
#62862=ORIENTED_EDGE('',*,*,#47282,.F.);
#62863=ORIENTED_EDGE('',*,*,#47297,.T.);
#62864=ORIENTED_EDGE('',*,*,#47284,.F.);
#62865=ORIENTED_EDGE('',*,*,#47298,.T.);
#62866=ORIENTED_EDGE('',*,*,#47278,.F.);
#62867=ORIENTED_EDGE('',*,*,#47299,.T.);
#62868=ORIENTED_EDGE('',*,*,#47280,.F.);
#62869=ORIENTED_EDGE('',*,*,#47300,.T.);
#62870=ORIENTED_EDGE('',*,*,#47301,.T.);
#62871=ORIENTED_EDGE('',*,*,#47302,.T.);
#62872=ORIENTED_EDGE('',*,*,#47303,.F.);
#62873=ORIENTED_EDGE('',*,*,#47304,.F.);
#62874=ORIENTED_EDGE('',*,*,#47305,.F.);
#62875=ORIENTED_EDGE('',*,*,#47306,.T.);
#62876=ORIENTED_EDGE('',*,*,#47304,.T.);
#62877=ORIENTED_EDGE('',*,*,#47307,.T.);
#62878=ORIENTED_EDGE('',*,*,#47308,.T.);
#62879=ORIENTED_EDGE('',*,*,#47309,.T.);
#62880=ORIENTED_EDGE('',*,*,#47310,.T.);
#62881=ORIENTED_EDGE('',*,*,#47311,.T.);
#62882=ORIENTED_EDGE('',*,*,#47312,.T.);
#62883=ORIENTED_EDGE('',*,*,#47313,.T.);
#62884=ORIENTED_EDGE('',*,*,#47314,.T.);
#62885=ORIENTED_EDGE('',*,*,#47315,.T.);
#62886=ORIENTED_EDGE('',*,*,#47316,.F.);
#62887=ORIENTED_EDGE('',*,*,#47317,.F.);
#62888=ORIENTED_EDGE('',*,*,#47318,.F.);
#62889=ORIENTED_EDGE('',*,*,#47319,.T.);
#62890=ORIENTED_EDGE('',*,*,#47317,.T.);
#62891=ORIENTED_EDGE('',*,*,#47320,.T.);
#62892=ORIENTED_EDGE('',*,*,#47321,.T.);
#62893=ORIENTED_EDGE('',*,*,#47322,.T.);
#62894=ORIENTED_EDGE('',*,*,#46591,.F.);
#62895=ORIENTED_EDGE('',*,*,#47323,.T.);
#62896=ORIENTED_EDGE('',*,*,#47301,.F.);
#62897=ORIENTED_EDGE('',*,*,#47324,.T.);
#62898=ORIENTED_EDGE('',*,*,#47321,.F.);
#62899=ORIENTED_EDGE('',*,*,#47325,.T.);
#62900=ORIENTED_EDGE('',*,*,#46142,.F.);
#62901=ORIENTED_EDGE('',*,*,#47326,.T.);
#62902=ORIENTED_EDGE('',*,*,#47312,.F.);
#62903=ORIENTED_EDGE('',*,*,#47327,.T.);
#62904=ORIENTED_EDGE('',*,*,#47314,.F.);
#62905=ORIENTED_EDGE('',*,*,#47328,.T.);
#62906=ORIENTED_EDGE('',*,*,#47308,.F.);
#62907=ORIENTED_EDGE('',*,*,#47329,.T.);
#62908=ORIENTED_EDGE('',*,*,#47310,.F.);
#62909=ORIENTED_EDGE('',*,*,#47330,.T.);
#62910=ORIENTED_EDGE('',*,*,#47331,.T.);
#62911=ORIENTED_EDGE('',*,*,#47332,.T.);
#62912=ORIENTED_EDGE('',*,*,#47333,.F.);
#62913=ORIENTED_EDGE('',*,*,#47334,.F.);
#62914=ORIENTED_EDGE('',*,*,#47335,.F.);
#62915=ORIENTED_EDGE('',*,*,#47336,.T.);
#62916=ORIENTED_EDGE('',*,*,#47334,.T.);
#62917=ORIENTED_EDGE('',*,*,#47337,.T.);
#62918=ORIENTED_EDGE('',*,*,#47338,.T.);
#62919=ORIENTED_EDGE('',*,*,#47339,.T.);
#62920=ORIENTED_EDGE('',*,*,#47340,.T.);
#62921=ORIENTED_EDGE('',*,*,#47341,.T.);
#62922=ORIENTED_EDGE('',*,*,#47342,.T.);
#62923=ORIENTED_EDGE('',*,*,#47343,.T.);
#62924=ORIENTED_EDGE('',*,*,#47344,.T.);
#62925=ORIENTED_EDGE('',*,*,#47345,.T.);
#62926=ORIENTED_EDGE('',*,*,#47346,.F.);
#62927=ORIENTED_EDGE('',*,*,#47347,.F.);
#62928=ORIENTED_EDGE('',*,*,#47348,.F.);
#62929=ORIENTED_EDGE('',*,*,#47349,.T.);
#62930=ORIENTED_EDGE('',*,*,#47347,.T.);
#62931=ORIENTED_EDGE('',*,*,#47350,.T.);
#62932=ORIENTED_EDGE('',*,*,#47351,.T.);
#62933=ORIENTED_EDGE('',*,*,#47352,.T.);
#62934=ORIENTED_EDGE('',*,*,#46597,.F.);
#62935=ORIENTED_EDGE('',*,*,#47353,.T.);
#62936=ORIENTED_EDGE('',*,*,#47331,.F.);
#62937=ORIENTED_EDGE('',*,*,#47354,.T.);
#62938=ORIENTED_EDGE('',*,*,#47351,.F.);
#62939=ORIENTED_EDGE('',*,*,#47355,.T.);
#62940=ORIENTED_EDGE('',*,*,#46136,.F.);
#62941=ORIENTED_EDGE('',*,*,#47356,.T.);
#62942=ORIENTED_EDGE('',*,*,#47342,.F.);
#62943=ORIENTED_EDGE('',*,*,#47357,.T.);
#62944=ORIENTED_EDGE('',*,*,#47344,.F.);
#62945=ORIENTED_EDGE('',*,*,#47358,.T.);
#62946=ORIENTED_EDGE('',*,*,#47338,.F.);
#62947=ORIENTED_EDGE('',*,*,#47359,.T.);
#62948=ORIENTED_EDGE('',*,*,#47340,.F.);
#62949=ORIENTED_EDGE('',*,*,#47360,.T.);
#62950=ORIENTED_EDGE('',*,*,#47361,.T.);
#62951=ORIENTED_EDGE('',*,*,#47362,.T.);
#62952=ORIENTED_EDGE('',*,*,#47363,.F.);
#62953=ORIENTED_EDGE('',*,*,#47364,.F.);
#62954=ORIENTED_EDGE('',*,*,#47365,.F.);
#62955=ORIENTED_EDGE('',*,*,#47366,.T.);
#62956=ORIENTED_EDGE('',*,*,#47364,.T.);
#62957=ORIENTED_EDGE('',*,*,#47367,.T.);
#62958=ORIENTED_EDGE('',*,*,#47368,.T.);
#62959=ORIENTED_EDGE('',*,*,#47369,.T.);
#62960=ORIENTED_EDGE('',*,*,#47370,.T.);
#62961=ORIENTED_EDGE('',*,*,#47371,.T.);
#62962=ORIENTED_EDGE('',*,*,#47372,.T.);
#62963=ORIENTED_EDGE('',*,*,#47373,.T.);
#62964=ORIENTED_EDGE('',*,*,#47374,.T.);
#62965=ORIENTED_EDGE('',*,*,#47375,.T.);
#62966=ORIENTED_EDGE('',*,*,#47376,.F.);
#62967=ORIENTED_EDGE('',*,*,#47377,.F.);
#62968=ORIENTED_EDGE('',*,*,#47378,.F.);
#62969=ORIENTED_EDGE('',*,*,#47379,.T.);
#62970=ORIENTED_EDGE('',*,*,#47377,.T.);
#62971=ORIENTED_EDGE('',*,*,#47380,.T.);
#62972=ORIENTED_EDGE('',*,*,#47381,.T.);
#62973=ORIENTED_EDGE('',*,*,#47382,.T.);
#62974=ORIENTED_EDGE('',*,*,#46603,.F.);
#62975=ORIENTED_EDGE('',*,*,#47383,.T.);
#62976=ORIENTED_EDGE('',*,*,#47361,.F.);
#62977=ORIENTED_EDGE('',*,*,#47384,.T.);
#62978=ORIENTED_EDGE('',*,*,#47381,.F.);
#62979=ORIENTED_EDGE('',*,*,#47385,.T.);
#62980=ORIENTED_EDGE('',*,*,#46130,.F.);
#62981=ORIENTED_EDGE('',*,*,#47386,.T.);
#62982=ORIENTED_EDGE('',*,*,#47372,.F.);
#62983=ORIENTED_EDGE('',*,*,#47387,.T.);
#62984=ORIENTED_EDGE('',*,*,#47374,.F.);
#62985=ORIENTED_EDGE('',*,*,#47388,.T.);
#62986=ORIENTED_EDGE('',*,*,#47368,.F.);
#62987=ORIENTED_EDGE('',*,*,#47389,.T.);
#62988=ORIENTED_EDGE('',*,*,#47370,.F.);
#62989=ORIENTED_EDGE('',*,*,#47390,.T.);
#62990=ORIENTED_EDGE('',*,*,#47391,.T.);
#62991=ORIENTED_EDGE('',*,*,#47392,.T.);
#62992=ORIENTED_EDGE('',*,*,#47393,.F.);
#62993=ORIENTED_EDGE('',*,*,#47394,.F.);
#62994=ORIENTED_EDGE('',*,*,#47395,.F.);
#62995=ORIENTED_EDGE('',*,*,#47396,.T.);
#62996=ORIENTED_EDGE('',*,*,#47394,.T.);
#62997=ORIENTED_EDGE('',*,*,#47397,.T.);
#62998=ORIENTED_EDGE('',*,*,#47398,.T.);
#62999=ORIENTED_EDGE('',*,*,#47399,.T.);
#63000=ORIENTED_EDGE('',*,*,#47400,.T.);
#63001=ORIENTED_EDGE('',*,*,#47401,.T.);
#63002=ORIENTED_EDGE('',*,*,#47402,.T.);
#63003=ORIENTED_EDGE('',*,*,#47403,.T.);
#63004=ORIENTED_EDGE('',*,*,#47404,.T.);
#63005=ORIENTED_EDGE('',*,*,#47405,.T.);
#63006=ORIENTED_EDGE('',*,*,#47406,.F.);
#63007=ORIENTED_EDGE('',*,*,#47407,.F.);
#63008=ORIENTED_EDGE('',*,*,#47408,.F.);
#63009=ORIENTED_EDGE('',*,*,#47409,.T.);
#63010=ORIENTED_EDGE('',*,*,#47407,.T.);
#63011=ORIENTED_EDGE('',*,*,#47410,.T.);
#63012=ORIENTED_EDGE('',*,*,#47411,.T.);
#63013=ORIENTED_EDGE('',*,*,#47412,.T.);
#63014=ORIENTED_EDGE('',*,*,#46609,.F.);
#63015=ORIENTED_EDGE('',*,*,#47413,.T.);
#63016=ORIENTED_EDGE('',*,*,#47391,.F.);
#63017=ORIENTED_EDGE('',*,*,#47414,.T.);
#63018=ORIENTED_EDGE('',*,*,#47411,.F.);
#63019=ORIENTED_EDGE('',*,*,#47415,.T.);
#63020=ORIENTED_EDGE('',*,*,#46124,.F.);
#63021=ORIENTED_EDGE('',*,*,#47416,.T.);
#63022=ORIENTED_EDGE('',*,*,#47402,.F.);
#63023=ORIENTED_EDGE('',*,*,#47417,.T.);
#63024=ORIENTED_EDGE('',*,*,#47404,.F.);
#63025=ORIENTED_EDGE('',*,*,#47418,.T.);
#63026=ORIENTED_EDGE('',*,*,#47398,.F.);
#63027=ORIENTED_EDGE('',*,*,#47419,.T.);
#63028=ORIENTED_EDGE('',*,*,#47400,.F.);
#63029=ORIENTED_EDGE('',*,*,#47420,.T.);
#63030=ORIENTED_EDGE('',*,*,#47421,.T.);
#63031=ORIENTED_EDGE('',*,*,#47422,.T.);
#63032=ORIENTED_EDGE('',*,*,#47423,.F.);
#63033=ORIENTED_EDGE('',*,*,#47424,.F.);
#63034=ORIENTED_EDGE('',*,*,#47425,.F.);
#63035=ORIENTED_EDGE('',*,*,#47426,.T.);
#63036=ORIENTED_EDGE('',*,*,#47424,.T.);
#63037=ORIENTED_EDGE('',*,*,#47427,.T.);
#63038=ORIENTED_EDGE('',*,*,#47428,.T.);
#63039=ORIENTED_EDGE('',*,*,#47429,.T.);
#63040=ORIENTED_EDGE('',*,*,#47430,.T.);
#63041=ORIENTED_EDGE('',*,*,#47431,.T.);
#63042=ORIENTED_EDGE('',*,*,#47432,.T.);
#63043=ORIENTED_EDGE('',*,*,#47433,.T.);
#63044=ORIENTED_EDGE('',*,*,#47434,.T.);
#63045=ORIENTED_EDGE('',*,*,#47435,.T.);
#63046=ORIENTED_EDGE('',*,*,#47436,.F.);
#63047=ORIENTED_EDGE('',*,*,#47437,.F.);
#63048=ORIENTED_EDGE('',*,*,#47438,.F.);
#63049=ORIENTED_EDGE('',*,*,#47439,.T.);
#63050=ORIENTED_EDGE('',*,*,#47437,.T.);
#63051=ORIENTED_EDGE('',*,*,#47440,.T.);
#63052=ORIENTED_EDGE('',*,*,#47441,.T.);
#63053=ORIENTED_EDGE('',*,*,#47442,.T.);
#63054=ORIENTED_EDGE('',*,*,#46615,.F.);
#63055=ORIENTED_EDGE('',*,*,#47443,.T.);
#63056=ORIENTED_EDGE('',*,*,#47421,.F.);
#63057=ORIENTED_EDGE('',*,*,#47444,.T.);
#63058=ORIENTED_EDGE('',*,*,#47441,.F.);
#63059=ORIENTED_EDGE('',*,*,#47445,.T.);
#63060=ORIENTED_EDGE('',*,*,#46118,.F.);
#63061=ORIENTED_EDGE('',*,*,#47446,.T.);
#63062=ORIENTED_EDGE('',*,*,#47432,.F.);
#63063=ORIENTED_EDGE('',*,*,#47447,.T.);
#63064=ORIENTED_EDGE('',*,*,#47434,.F.);
#63065=ORIENTED_EDGE('',*,*,#47448,.T.);
#63066=ORIENTED_EDGE('',*,*,#47428,.F.);
#63067=ORIENTED_EDGE('',*,*,#47449,.T.);
#63068=ORIENTED_EDGE('',*,*,#47430,.F.);
#63069=ORIENTED_EDGE('',*,*,#47450,.T.);
#63070=ORIENTED_EDGE('',*,*,#47451,.T.);
#63071=ORIENTED_EDGE('',*,*,#47452,.T.);
#63072=ORIENTED_EDGE('',*,*,#47453,.F.);
#63073=ORIENTED_EDGE('',*,*,#47454,.F.);
#63074=ORIENTED_EDGE('',*,*,#47455,.F.);
#63075=ORIENTED_EDGE('',*,*,#47456,.T.);
#63076=ORIENTED_EDGE('',*,*,#47454,.T.);
#63077=ORIENTED_EDGE('',*,*,#47457,.T.);
#63078=ORIENTED_EDGE('',*,*,#47458,.T.);
#63079=ORIENTED_EDGE('',*,*,#47459,.T.);
#63080=ORIENTED_EDGE('',*,*,#47460,.T.);
#63081=ORIENTED_EDGE('',*,*,#47461,.T.);
#63082=ORIENTED_EDGE('',*,*,#47462,.T.);
#63083=ORIENTED_EDGE('',*,*,#47463,.T.);
#63084=ORIENTED_EDGE('',*,*,#47464,.T.);
#63085=ORIENTED_EDGE('',*,*,#47465,.T.);
#63086=ORIENTED_EDGE('',*,*,#47466,.F.);
#63087=ORIENTED_EDGE('',*,*,#47467,.F.);
#63088=ORIENTED_EDGE('',*,*,#47468,.F.);
#63089=ORIENTED_EDGE('',*,*,#47469,.T.);
#63090=ORIENTED_EDGE('',*,*,#47467,.T.);
#63091=ORIENTED_EDGE('',*,*,#47470,.T.);
#63092=ORIENTED_EDGE('',*,*,#47471,.T.);
#63093=ORIENTED_EDGE('',*,*,#47472,.T.);
#63094=ORIENTED_EDGE('',*,*,#46621,.F.);
#63095=ORIENTED_EDGE('',*,*,#47473,.T.);
#63096=ORIENTED_EDGE('',*,*,#47451,.F.);
#63097=ORIENTED_EDGE('',*,*,#47474,.T.);
#63098=ORIENTED_EDGE('',*,*,#47471,.F.);
#63099=ORIENTED_EDGE('',*,*,#47475,.T.);
#63100=ORIENTED_EDGE('',*,*,#46112,.F.);
#63101=ORIENTED_EDGE('',*,*,#47476,.T.);
#63102=ORIENTED_EDGE('',*,*,#47462,.F.);
#63103=ORIENTED_EDGE('',*,*,#47477,.T.);
#63104=ORIENTED_EDGE('',*,*,#47464,.F.);
#63105=ORIENTED_EDGE('',*,*,#47478,.T.);
#63106=ORIENTED_EDGE('',*,*,#47458,.F.);
#63107=ORIENTED_EDGE('',*,*,#47479,.T.);
#63108=ORIENTED_EDGE('',*,*,#47460,.F.);
#63109=ORIENTED_EDGE('',*,*,#47480,.T.);
#63110=ORIENTED_EDGE('',*,*,#47481,.T.);
#63111=ORIENTED_EDGE('',*,*,#47482,.T.);
#63112=ORIENTED_EDGE('',*,*,#47483,.F.);
#63113=ORIENTED_EDGE('',*,*,#47484,.F.);
#63114=ORIENTED_EDGE('',*,*,#47485,.F.);
#63115=ORIENTED_EDGE('',*,*,#47486,.T.);
#63116=ORIENTED_EDGE('',*,*,#47484,.T.);
#63117=ORIENTED_EDGE('',*,*,#47487,.T.);
#63118=ORIENTED_EDGE('',*,*,#47488,.T.);
#63119=ORIENTED_EDGE('',*,*,#47489,.T.);
#63120=ORIENTED_EDGE('',*,*,#47490,.T.);
#63121=ORIENTED_EDGE('',*,*,#47491,.T.);
#63122=ORIENTED_EDGE('',*,*,#47492,.T.);
#63123=ORIENTED_EDGE('',*,*,#47493,.T.);
#63124=ORIENTED_EDGE('',*,*,#47494,.T.);
#63125=ORIENTED_EDGE('',*,*,#47495,.T.);
#63126=ORIENTED_EDGE('',*,*,#47496,.F.);
#63127=ORIENTED_EDGE('',*,*,#47497,.F.);
#63128=ORIENTED_EDGE('',*,*,#47498,.F.);
#63129=ORIENTED_EDGE('',*,*,#47499,.T.);
#63130=ORIENTED_EDGE('',*,*,#47497,.T.);
#63131=ORIENTED_EDGE('',*,*,#47500,.T.);
#63132=ORIENTED_EDGE('',*,*,#47501,.T.);
#63133=ORIENTED_EDGE('',*,*,#47502,.T.);
#63134=ORIENTED_EDGE('',*,*,#46627,.F.);
#63135=ORIENTED_EDGE('',*,*,#47503,.T.);
#63136=ORIENTED_EDGE('',*,*,#47481,.F.);
#63137=ORIENTED_EDGE('',*,*,#47504,.T.);
#63138=ORIENTED_EDGE('',*,*,#47501,.F.);
#63139=ORIENTED_EDGE('',*,*,#47505,.T.);
#63140=ORIENTED_EDGE('',*,*,#46106,.F.);
#63141=ORIENTED_EDGE('',*,*,#47506,.T.);
#63142=ORIENTED_EDGE('',*,*,#47492,.F.);
#63143=ORIENTED_EDGE('',*,*,#47507,.T.);
#63144=ORIENTED_EDGE('',*,*,#47494,.F.);
#63145=ORIENTED_EDGE('',*,*,#47508,.T.);
#63146=ORIENTED_EDGE('',*,*,#47488,.F.);
#63147=ORIENTED_EDGE('',*,*,#47509,.T.);
#63148=ORIENTED_EDGE('',*,*,#47490,.F.);
#63149=ORIENTED_EDGE('',*,*,#47510,.T.);
#63150=ORIENTED_EDGE('',*,*,#47511,.T.);
#63151=ORIENTED_EDGE('',*,*,#47512,.T.);
#63152=ORIENTED_EDGE('',*,*,#47513,.F.);
#63153=ORIENTED_EDGE('',*,*,#47514,.F.);
#63154=ORIENTED_EDGE('',*,*,#47515,.F.);
#63155=ORIENTED_EDGE('',*,*,#47516,.T.);
#63156=ORIENTED_EDGE('',*,*,#47514,.T.);
#63157=ORIENTED_EDGE('',*,*,#47517,.T.);
#63158=ORIENTED_EDGE('',*,*,#47518,.T.);
#63159=ORIENTED_EDGE('',*,*,#47519,.T.);
#63160=ORIENTED_EDGE('',*,*,#47520,.T.);
#63161=ORIENTED_EDGE('',*,*,#47521,.T.);
#63162=ORIENTED_EDGE('',*,*,#47522,.T.);
#63163=ORIENTED_EDGE('',*,*,#47523,.T.);
#63164=ORIENTED_EDGE('',*,*,#47524,.T.);
#63165=ORIENTED_EDGE('',*,*,#47525,.T.);
#63166=ORIENTED_EDGE('',*,*,#47526,.F.);
#63167=ORIENTED_EDGE('',*,*,#47527,.F.);
#63168=ORIENTED_EDGE('',*,*,#47528,.F.);
#63169=ORIENTED_EDGE('',*,*,#47529,.T.);
#63170=ORIENTED_EDGE('',*,*,#47527,.T.);
#63171=ORIENTED_EDGE('',*,*,#47530,.T.);
#63172=ORIENTED_EDGE('',*,*,#47531,.T.);
#63173=ORIENTED_EDGE('',*,*,#47532,.T.);
#63174=ORIENTED_EDGE('',*,*,#46633,.F.);
#63175=ORIENTED_EDGE('',*,*,#47533,.T.);
#63176=ORIENTED_EDGE('',*,*,#47511,.F.);
#63177=ORIENTED_EDGE('',*,*,#47534,.T.);
#63178=ORIENTED_EDGE('',*,*,#47531,.F.);
#63179=ORIENTED_EDGE('',*,*,#47535,.T.);
#63180=ORIENTED_EDGE('',*,*,#46100,.F.);
#63181=ORIENTED_EDGE('',*,*,#47536,.T.);
#63182=ORIENTED_EDGE('',*,*,#47522,.F.);
#63183=ORIENTED_EDGE('',*,*,#47537,.T.);
#63184=ORIENTED_EDGE('',*,*,#47524,.F.);
#63185=ORIENTED_EDGE('',*,*,#47538,.T.);
#63186=ORIENTED_EDGE('',*,*,#47518,.F.);
#63187=ORIENTED_EDGE('',*,*,#47539,.T.);
#63188=ORIENTED_EDGE('',*,*,#47520,.F.);
#63189=ORIENTED_EDGE('',*,*,#47540,.T.);
#63190=ORIENTED_EDGE('',*,*,#47541,.T.);
#63191=ORIENTED_EDGE('',*,*,#47542,.T.);
#63192=ORIENTED_EDGE('',*,*,#47543,.F.);
#63193=ORIENTED_EDGE('',*,*,#47544,.F.);
#63194=ORIENTED_EDGE('',*,*,#47545,.F.);
#63195=ORIENTED_EDGE('',*,*,#47546,.T.);
#63196=ORIENTED_EDGE('',*,*,#47544,.T.);
#63197=ORIENTED_EDGE('',*,*,#47547,.T.);
#63198=ORIENTED_EDGE('',*,*,#47548,.T.);
#63199=ORIENTED_EDGE('',*,*,#47549,.T.);
#63200=ORIENTED_EDGE('',*,*,#47550,.T.);
#63201=ORIENTED_EDGE('',*,*,#47551,.T.);
#63202=ORIENTED_EDGE('',*,*,#47552,.T.);
#63203=ORIENTED_EDGE('',*,*,#47553,.T.);
#63204=ORIENTED_EDGE('',*,*,#47554,.T.);
#63205=ORIENTED_EDGE('',*,*,#47555,.T.);
#63206=ORIENTED_EDGE('',*,*,#47556,.F.);
#63207=ORIENTED_EDGE('',*,*,#47557,.F.);
#63208=ORIENTED_EDGE('',*,*,#47558,.F.);
#63209=ORIENTED_EDGE('',*,*,#47559,.T.);
#63210=ORIENTED_EDGE('',*,*,#47557,.T.);
#63211=ORIENTED_EDGE('',*,*,#47560,.T.);
#63212=ORIENTED_EDGE('',*,*,#47561,.T.);
#63213=ORIENTED_EDGE('',*,*,#47562,.T.);
#63214=ORIENTED_EDGE('',*,*,#46278,.F.);
#63215=ORIENTED_EDGE('',*,*,#47563,.T.);
#63216=ORIENTED_EDGE('',*,*,#47541,.F.);
#63217=ORIENTED_EDGE('',*,*,#47564,.T.);
#63218=ORIENTED_EDGE('',*,*,#47561,.F.);
#63219=ORIENTED_EDGE('',*,*,#47565,.T.);
#63220=ORIENTED_EDGE('',*,*,#46094,.F.);
#63221=ORIENTED_EDGE('',*,*,#47566,.T.);
#63222=ORIENTED_EDGE('',*,*,#47552,.F.);
#63223=ORIENTED_EDGE('',*,*,#47567,.T.);
#63224=ORIENTED_EDGE('',*,*,#47554,.F.);
#63225=ORIENTED_EDGE('',*,*,#47568,.T.);
#63226=ORIENTED_EDGE('',*,*,#47548,.F.);
#63227=ORIENTED_EDGE('',*,*,#47569,.T.);
#63228=ORIENTED_EDGE('',*,*,#47550,.F.);
#63229=ORIENTED_EDGE('',*,*,#47570,.T.);
#63230=ORIENTED_EDGE('',*,*,#47571,.T.);
#63231=ORIENTED_EDGE('',*,*,#47572,.T.);
#63232=ORIENTED_EDGE('',*,*,#47573,.F.);
#63233=ORIENTED_EDGE('',*,*,#47574,.F.);
#63234=ORIENTED_EDGE('',*,*,#47575,.F.);
#63235=ORIENTED_EDGE('',*,*,#47576,.T.);
#63236=ORIENTED_EDGE('',*,*,#47574,.T.);
#63237=ORIENTED_EDGE('',*,*,#47577,.T.);
#63238=ORIENTED_EDGE('',*,*,#47578,.T.);
#63239=ORIENTED_EDGE('',*,*,#47579,.T.);
#63240=ORIENTED_EDGE('',*,*,#47580,.T.);
#63241=ORIENTED_EDGE('',*,*,#47581,.T.);
#63242=ORIENTED_EDGE('',*,*,#47582,.T.);
#63243=ORIENTED_EDGE('',*,*,#47583,.T.);
#63244=ORIENTED_EDGE('',*,*,#47584,.T.);
#63245=ORIENTED_EDGE('',*,*,#47585,.T.);
#63246=ORIENTED_EDGE('',*,*,#47586,.F.);
#63247=ORIENTED_EDGE('',*,*,#47587,.F.);
#63248=ORIENTED_EDGE('',*,*,#47588,.F.);
#63249=ORIENTED_EDGE('',*,*,#47589,.T.);
#63250=ORIENTED_EDGE('',*,*,#47587,.T.);
#63251=ORIENTED_EDGE('',*,*,#47590,.T.);
#63252=ORIENTED_EDGE('',*,*,#47591,.T.);
#63253=ORIENTED_EDGE('',*,*,#47592,.T.);
#63254=ORIENTED_EDGE('',*,*,#46284,.F.);
#63255=ORIENTED_EDGE('',*,*,#47593,.T.);
#63256=ORIENTED_EDGE('',*,*,#47571,.F.);
#63257=ORIENTED_EDGE('',*,*,#47594,.T.);
#63258=ORIENTED_EDGE('',*,*,#47591,.F.);
#63259=ORIENTED_EDGE('',*,*,#47595,.T.);
#63260=ORIENTED_EDGE('',*,*,#46088,.F.);
#63261=ORIENTED_EDGE('',*,*,#47596,.T.);
#63262=ORIENTED_EDGE('',*,*,#47582,.F.);
#63263=ORIENTED_EDGE('',*,*,#47597,.T.);
#63264=ORIENTED_EDGE('',*,*,#47584,.F.);
#63265=ORIENTED_EDGE('',*,*,#47598,.T.);
#63266=ORIENTED_EDGE('',*,*,#47578,.F.);
#63267=ORIENTED_EDGE('',*,*,#47599,.T.);
#63268=ORIENTED_EDGE('',*,*,#47580,.F.);
#63269=ORIENTED_EDGE('',*,*,#47600,.T.);
#63270=ORIENTED_EDGE('',*,*,#47601,.T.);
#63271=ORIENTED_EDGE('',*,*,#47602,.T.);
#63272=ORIENTED_EDGE('',*,*,#47603,.F.);
#63273=ORIENTED_EDGE('',*,*,#47604,.F.);
#63274=ORIENTED_EDGE('',*,*,#47605,.F.);
#63275=ORIENTED_EDGE('',*,*,#47606,.T.);
#63276=ORIENTED_EDGE('',*,*,#47604,.T.);
#63277=ORIENTED_EDGE('',*,*,#47607,.T.);
#63278=ORIENTED_EDGE('',*,*,#47608,.T.);
#63279=ORIENTED_EDGE('',*,*,#47609,.T.);
#63280=ORIENTED_EDGE('',*,*,#47610,.T.);
#63281=ORIENTED_EDGE('',*,*,#47611,.T.);
#63282=ORIENTED_EDGE('',*,*,#47612,.T.);
#63283=ORIENTED_EDGE('',*,*,#47613,.T.);
#63284=ORIENTED_EDGE('',*,*,#47614,.T.);
#63285=ORIENTED_EDGE('',*,*,#47615,.T.);
#63286=ORIENTED_EDGE('',*,*,#47616,.F.);
#63287=ORIENTED_EDGE('',*,*,#47617,.F.);
#63288=ORIENTED_EDGE('',*,*,#47618,.F.);
#63289=ORIENTED_EDGE('',*,*,#47619,.T.);
#63290=ORIENTED_EDGE('',*,*,#47617,.T.);
#63291=ORIENTED_EDGE('',*,*,#47620,.T.);
#63292=ORIENTED_EDGE('',*,*,#47621,.T.);
#63293=ORIENTED_EDGE('',*,*,#47622,.T.);
#63294=ORIENTED_EDGE('',*,*,#46290,.F.);
#63295=ORIENTED_EDGE('',*,*,#47623,.T.);
#63296=ORIENTED_EDGE('',*,*,#47601,.F.);
#63297=ORIENTED_EDGE('',*,*,#47624,.T.);
#63298=ORIENTED_EDGE('',*,*,#47621,.F.);
#63299=ORIENTED_EDGE('',*,*,#47625,.T.);
#63300=ORIENTED_EDGE('',*,*,#46082,.F.);
#63301=ORIENTED_EDGE('',*,*,#47626,.T.);
#63302=ORIENTED_EDGE('',*,*,#47612,.F.);
#63303=ORIENTED_EDGE('',*,*,#47627,.T.);
#63304=ORIENTED_EDGE('',*,*,#47614,.F.);
#63305=ORIENTED_EDGE('',*,*,#47628,.T.);
#63306=ORIENTED_EDGE('',*,*,#47608,.F.);
#63307=ORIENTED_EDGE('',*,*,#47629,.T.);
#63308=ORIENTED_EDGE('',*,*,#47610,.F.);
#63309=ORIENTED_EDGE('',*,*,#47630,.T.);
#63310=ORIENTED_EDGE('',*,*,#47631,.T.);
#63311=ORIENTED_EDGE('',*,*,#47632,.T.);
#63312=ORIENTED_EDGE('',*,*,#47633,.F.);
#63313=ORIENTED_EDGE('',*,*,#47634,.F.);
#63314=ORIENTED_EDGE('',*,*,#47635,.F.);
#63315=ORIENTED_EDGE('',*,*,#47636,.T.);
#63316=ORIENTED_EDGE('',*,*,#47634,.T.);
#63317=ORIENTED_EDGE('',*,*,#47637,.T.);
#63318=ORIENTED_EDGE('',*,*,#47638,.T.);
#63319=ORIENTED_EDGE('',*,*,#47639,.T.);
#63320=ORIENTED_EDGE('',*,*,#47640,.T.);
#63321=ORIENTED_EDGE('',*,*,#47641,.T.);
#63322=ORIENTED_EDGE('',*,*,#47642,.T.);
#63323=ORIENTED_EDGE('',*,*,#47643,.T.);
#63324=ORIENTED_EDGE('',*,*,#47644,.T.);
#63325=ORIENTED_EDGE('',*,*,#47645,.T.);
#63326=ORIENTED_EDGE('',*,*,#47646,.F.);
#63327=ORIENTED_EDGE('',*,*,#47647,.F.);
#63328=ORIENTED_EDGE('',*,*,#47648,.F.);
#63329=ORIENTED_EDGE('',*,*,#47649,.T.);
#63330=ORIENTED_EDGE('',*,*,#47647,.T.);
#63331=ORIENTED_EDGE('',*,*,#47650,.T.);
#63332=ORIENTED_EDGE('',*,*,#47651,.T.);
#63333=ORIENTED_EDGE('',*,*,#47652,.T.);
#63334=ORIENTED_EDGE('',*,*,#46296,.F.);
#63335=ORIENTED_EDGE('',*,*,#47653,.T.);
#63336=ORIENTED_EDGE('',*,*,#47631,.F.);
#63337=ORIENTED_EDGE('',*,*,#47654,.T.);
#63338=ORIENTED_EDGE('',*,*,#47651,.F.);
#63339=ORIENTED_EDGE('',*,*,#47655,.T.);
#63340=ORIENTED_EDGE('',*,*,#46076,.F.);
#63341=ORIENTED_EDGE('',*,*,#47656,.T.);
#63342=ORIENTED_EDGE('',*,*,#47642,.F.);
#63343=ORIENTED_EDGE('',*,*,#47657,.T.);
#63344=ORIENTED_EDGE('',*,*,#47644,.F.);
#63345=ORIENTED_EDGE('',*,*,#47658,.T.);
#63346=ORIENTED_EDGE('',*,*,#47638,.F.);
#63347=ORIENTED_EDGE('',*,*,#47659,.T.);
#63348=ORIENTED_EDGE('',*,*,#47640,.F.);
#63349=ORIENTED_EDGE('',*,*,#47660,.T.);
#63350=ORIENTED_EDGE('',*,*,#47661,.T.);
#63351=ORIENTED_EDGE('',*,*,#47662,.T.);
#63352=ORIENTED_EDGE('',*,*,#47663,.F.);
#63353=ORIENTED_EDGE('',*,*,#47664,.F.);
#63354=ORIENTED_EDGE('',*,*,#47665,.F.);
#63355=ORIENTED_EDGE('',*,*,#47666,.T.);
#63356=ORIENTED_EDGE('',*,*,#47664,.T.);
#63357=ORIENTED_EDGE('',*,*,#47667,.T.);
#63358=ORIENTED_EDGE('',*,*,#47668,.T.);
#63359=ORIENTED_EDGE('',*,*,#47669,.T.);
#63360=ORIENTED_EDGE('',*,*,#47670,.T.);
#63361=ORIENTED_EDGE('',*,*,#47671,.T.);
#63362=ORIENTED_EDGE('',*,*,#47672,.T.);
#63363=ORIENTED_EDGE('',*,*,#47673,.T.);
#63364=ORIENTED_EDGE('',*,*,#47674,.T.);
#63365=ORIENTED_EDGE('',*,*,#47675,.T.);
#63366=ORIENTED_EDGE('',*,*,#47676,.F.);
#63367=ORIENTED_EDGE('',*,*,#47677,.F.);
#63368=ORIENTED_EDGE('',*,*,#47678,.F.);
#63369=ORIENTED_EDGE('',*,*,#47679,.T.);
#63370=ORIENTED_EDGE('',*,*,#47677,.T.);
#63371=ORIENTED_EDGE('',*,*,#47680,.T.);
#63372=ORIENTED_EDGE('',*,*,#47681,.T.);
#63373=ORIENTED_EDGE('',*,*,#47682,.T.);
#63374=ORIENTED_EDGE('',*,*,#46302,.F.);
#63375=ORIENTED_EDGE('',*,*,#47683,.T.);
#63376=ORIENTED_EDGE('',*,*,#47661,.F.);
#63377=ORIENTED_EDGE('',*,*,#47684,.T.);
#63378=ORIENTED_EDGE('',*,*,#47681,.F.);
#63379=ORIENTED_EDGE('',*,*,#47685,.T.);
#63380=ORIENTED_EDGE('',*,*,#46070,.F.);
#63381=ORIENTED_EDGE('',*,*,#47686,.T.);
#63382=ORIENTED_EDGE('',*,*,#47672,.F.);
#63383=ORIENTED_EDGE('',*,*,#47687,.T.);
#63384=ORIENTED_EDGE('',*,*,#47674,.F.);
#63385=ORIENTED_EDGE('',*,*,#47688,.T.);
#63386=ORIENTED_EDGE('',*,*,#47668,.F.);
#63387=ORIENTED_EDGE('',*,*,#47689,.T.);
#63388=ORIENTED_EDGE('',*,*,#47670,.F.);
#63389=ORIENTED_EDGE('',*,*,#47690,.T.);
#63390=ORIENTED_EDGE('',*,*,#47691,.T.);
#63391=ORIENTED_EDGE('',*,*,#47692,.T.);
#63392=ORIENTED_EDGE('',*,*,#47693,.F.);
#63393=ORIENTED_EDGE('',*,*,#47694,.F.);
#63394=ORIENTED_EDGE('',*,*,#47695,.F.);
#63395=ORIENTED_EDGE('',*,*,#47696,.T.);
#63396=ORIENTED_EDGE('',*,*,#47694,.T.);
#63397=ORIENTED_EDGE('',*,*,#47697,.T.);
#63398=ORIENTED_EDGE('',*,*,#47698,.T.);
#63399=ORIENTED_EDGE('',*,*,#47699,.T.);
#63400=ORIENTED_EDGE('',*,*,#47700,.T.);
#63401=ORIENTED_EDGE('',*,*,#47701,.T.);
#63402=ORIENTED_EDGE('',*,*,#47702,.T.);
#63403=ORIENTED_EDGE('',*,*,#47703,.T.);
#63404=ORIENTED_EDGE('',*,*,#47704,.T.);
#63405=ORIENTED_EDGE('',*,*,#47705,.T.);
#63406=ORIENTED_EDGE('',*,*,#47706,.F.);
#63407=ORIENTED_EDGE('',*,*,#47707,.F.);
#63408=ORIENTED_EDGE('',*,*,#47708,.F.);
#63409=ORIENTED_EDGE('',*,*,#47709,.T.);
#63410=ORIENTED_EDGE('',*,*,#47707,.T.);
#63411=ORIENTED_EDGE('',*,*,#47710,.T.);
#63412=ORIENTED_EDGE('',*,*,#47711,.T.);
#63413=ORIENTED_EDGE('',*,*,#47712,.T.);
#63414=ORIENTED_EDGE('',*,*,#46308,.F.);
#63415=ORIENTED_EDGE('',*,*,#47713,.T.);
#63416=ORIENTED_EDGE('',*,*,#47691,.F.);
#63417=ORIENTED_EDGE('',*,*,#47714,.T.);
#63418=ORIENTED_EDGE('',*,*,#47711,.F.);
#63419=ORIENTED_EDGE('',*,*,#47715,.T.);
#63420=ORIENTED_EDGE('',*,*,#46064,.F.);
#63421=ORIENTED_EDGE('',*,*,#47716,.T.);
#63422=ORIENTED_EDGE('',*,*,#47702,.F.);
#63423=ORIENTED_EDGE('',*,*,#47717,.T.);
#63424=ORIENTED_EDGE('',*,*,#47704,.F.);
#63425=ORIENTED_EDGE('',*,*,#47718,.T.);
#63426=ORIENTED_EDGE('',*,*,#47698,.F.);
#63427=ORIENTED_EDGE('',*,*,#47719,.T.);
#63428=ORIENTED_EDGE('',*,*,#47700,.F.);
#63429=ORIENTED_EDGE('',*,*,#47720,.T.);
#63430=ORIENTED_EDGE('',*,*,#47721,.T.);
#63431=ORIENTED_EDGE('',*,*,#47722,.T.);
#63432=ORIENTED_EDGE('',*,*,#47723,.F.);
#63433=ORIENTED_EDGE('',*,*,#47724,.F.);
#63434=ORIENTED_EDGE('',*,*,#47725,.F.);
#63435=ORIENTED_EDGE('',*,*,#47726,.T.);
#63436=ORIENTED_EDGE('',*,*,#47724,.T.);
#63437=ORIENTED_EDGE('',*,*,#47727,.T.);
#63438=ORIENTED_EDGE('',*,*,#47728,.T.);
#63439=ORIENTED_EDGE('',*,*,#47729,.T.);
#63440=ORIENTED_EDGE('',*,*,#47730,.T.);
#63441=ORIENTED_EDGE('',*,*,#47731,.T.);
#63442=ORIENTED_EDGE('',*,*,#47732,.T.);
#63443=ORIENTED_EDGE('',*,*,#47733,.T.);
#63444=ORIENTED_EDGE('',*,*,#47734,.T.);
#63445=ORIENTED_EDGE('',*,*,#47735,.T.);
#63446=ORIENTED_EDGE('',*,*,#47736,.F.);
#63447=ORIENTED_EDGE('',*,*,#47737,.F.);
#63448=ORIENTED_EDGE('',*,*,#47738,.F.);
#63449=ORIENTED_EDGE('',*,*,#47739,.T.);
#63450=ORIENTED_EDGE('',*,*,#47737,.T.);
#63451=ORIENTED_EDGE('',*,*,#47740,.T.);
#63452=ORIENTED_EDGE('',*,*,#47741,.T.);
#63453=ORIENTED_EDGE('',*,*,#47742,.T.);
#63454=ORIENTED_EDGE('',*,*,#46314,.F.);
#63455=ORIENTED_EDGE('',*,*,#47743,.T.);
#63456=ORIENTED_EDGE('',*,*,#47721,.F.);
#63457=ORIENTED_EDGE('',*,*,#47744,.T.);
#63458=ORIENTED_EDGE('',*,*,#47741,.F.);
#63459=ORIENTED_EDGE('',*,*,#47745,.T.);
#63460=ORIENTED_EDGE('',*,*,#46058,.F.);
#63461=ORIENTED_EDGE('',*,*,#47746,.T.);
#63462=ORIENTED_EDGE('',*,*,#47732,.F.);
#63463=ORIENTED_EDGE('',*,*,#47747,.T.);
#63464=ORIENTED_EDGE('',*,*,#47734,.F.);
#63465=ORIENTED_EDGE('',*,*,#47748,.T.);
#63466=ORIENTED_EDGE('',*,*,#47728,.F.);
#63467=ORIENTED_EDGE('',*,*,#47749,.T.);
#63468=ORIENTED_EDGE('',*,*,#47730,.F.);
#63469=ORIENTED_EDGE('',*,*,#47750,.T.);
#63470=ORIENTED_EDGE('',*,*,#47751,.T.);
#63471=ORIENTED_EDGE('',*,*,#47752,.T.);
#63472=ORIENTED_EDGE('',*,*,#47753,.F.);
#63473=ORIENTED_EDGE('',*,*,#47754,.F.);
#63474=ORIENTED_EDGE('',*,*,#47755,.F.);
#63475=ORIENTED_EDGE('',*,*,#47756,.T.);
#63476=ORIENTED_EDGE('',*,*,#47754,.T.);
#63477=ORIENTED_EDGE('',*,*,#47757,.T.);
#63478=ORIENTED_EDGE('',*,*,#47758,.T.);
#63479=ORIENTED_EDGE('',*,*,#47759,.T.);
#63480=ORIENTED_EDGE('',*,*,#47760,.T.);
#63481=ORIENTED_EDGE('',*,*,#47761,.T.);
#63482=ORIENTED_EDGE('',*,*,#47762,.T.);
#63483=ORIENTED_EDGE('',*,*,#47763,.T.);
#63484=ORIENTED_EDGE('',*,*,#47764,.T.);
#63485=ORIENTED_EDGE('',*,*,#47765,.T.);
#63486=ORIENTED_EDGE('',*,*,#47766,.F.);
#63487=ORIENTED_EDGE('',*,*,#47767,.F.);
#63488=ORIENTED_EDGE('',*,*,#47768,.F.);
#63489=ORIENTED_EDGE('',*,*,#47769,.T.);
#63490=ORIENTED_EDGE('',*,*,#47767,.T.);
#63491=ORIENTED_EDGE('',*,*,#47770,.T.);
#63492=ORIENTED_EDGE('',*,*,#47771,.T.);
#63493=ORIENTED_EDGE('',*,*,#47772,.T.);
#63494=ORIENTED_EDGE('',*,*,#46320,.F.);
#63495=ORIENTED_EDGE('',*,*,#47773,.T.);
#63496=ORIENTED_EDGE('',*,*,#47751,.F.);
#63497=ORIENTED_EDGE('',*,*,#47774,.T.);
#63498=ORIENTED_EDGE('',*,*,#47771,.F.);
#63499=ORIENTED_EDGE('',*,*,#47775,.T.);
#63500=ORIENTED_EDGE('',*,*,#46052,.F.);
#63501=ORIENTED_EDGE('',*,*,#47776,.T.);
#63502=ORIENTED_EDGE('',*,*,#47762,.F.);
#63503=ORIENTED_EDGE('',*,*,#47777,.T.);
#63504=ORIENTED_EDGE('',*,*,#47764,.F.);
#63505=ORIENTED_EDGE('',*,*,#47778,.T.);
#63506=ORIENTED_EDGE('',*,*,#47758,.F.);
#63507=ORIENTED_EDGE('',*,*,#47779,.T.);
#63508=ORIENTED_EDGE('',*,*,#47760,.F.);
#63509=ORIENTED_EDGE('',*,*,#47780,.T.);
#63510=ORIENTED_EDGE('',*,*,#47781,.T.);
#63511=ORIENTED_EDGE('',*,*,#47782,.T.);
#63512=ORIENTED_EDGE('',*,*,#47783,.F.);
#63513=ORIENTED_EDGE('',*,*,#47784,.F.);
#63514=ORIENTED_EDGE('',*,*,#47785,.F.);
#63515=ORIENTED_EDGE('',*,*,#47786,.T.);
#63516=ORIENTED_EDGE('',*,*,#47784,.T.);
#63517=ORIENTED_EDGE('',*,*,#47787,.T.);
#63518=ORIENTED_EDGE('',*,*,#47788,.T.);
#63519=ORIENTED_EDGE('',*,*,#47789,.T.);
#63520=ORIENTED_EDGE('',*,*,#47790,.T.);
#63521=ORIENTED_EDGE('',*,*,#47791,.T.);
#63522=ORIENTED_EDGE('',*,*,#47792,.T.);
#63523=ORIENTED_EDGE('',*,*,#47793,.T.);
#63524=ORIENTED_EDGE('',*,*,#47794,.T.);
#63525=ORIENTED_EDGE('',*,*,#47795,.T.);
#63526=ORIENTED_EDGE('',*,*,#47796,.F.);
#63527=ORIENTED_EDGE('',*,*,#47797,.F.);
#63528=ORIENTED_EDGE('',*,*,#47798,.F.);
#63529=ORIENTED_EDGE('',*,*,#47799,.T.);
#63530=ORIENTED_EDGE('',*,*,#47797,.T.);
#63531=ORIENTED_EDGE('',*,*,#47800,.T.);
#63532=ORIENTED_EDGE('',*,*,#47801,.T.);
#63533=ORIENTED_EDGE('',*,*,#47802,.T.);
#63534=ORIENTED_EDGE('',*,*,#46326,.F.);
#63535=ORIENTED_EDGE('',*,*,#47803,.T.);
#63536=ORIENTED_EDGE('',*,*,#47781,.F.);
#63537=ORIENTED_EDGE('',*,*,#47804,.T.);
#63538=ORIENTED_EDGE('',*,*,#47801,.F.);
#63539=ORIENTED_EDGE('',*,*,#47805,.T.);
#63540=ORIENTED_EDGE('',*,*,#46046,.F.);
#63541=ORIENTED_EDGE('',*,*,#47806,.T.);
#63542=ORIENTED_EDGE('',*,*,#47792,.F.);
#63543=ORIENTED_EDGE('',*,*,#47807,.T.);
#63544=ORIENTED_EDGE('',*,*,#47794,.F.);
#63545=ORIENTED_EDGE('',*,*,#47808,.T.);
#63546=ORIENTED_EDGE('',*,*,#47788,.F.);
#63547=ORIENTED_EDGE('',*,*,#47809,.T.);
#63548=ORIENTED_EDGE('',*,*,#47790,.F.);
#63549=ORIENTED_EDGE('',*,*,#47810,.T.);
#63550=ORIENTED_EDGE('',*,*,#47811,.T.);
#63551=ORIENTED_EDGE('',*,*,#47812,.T.);
#63552=ORIENTED_EDGE('',*,*,#47813,.F.);
#63553=ORIENTED_EDGE('',*,*,#47814,.F.);
#63554=ORIENTED_EDGE('',*,*,#47815,.F.);
#63555=ORIENTED_EDGE('',*,*,#47816,.T.);
#63556=ORIENTED_EDGE('',*,*,#47814,.T.);
#63557=ORIENTED_EDGE('',*,*,#47817,.T.);
#63558=ORIENTED_EDGE('',*,*,#47818,.T.);
#63559=ORIENTED_EDGE('',*,*,#47819,.T.);
#63560=ORIENTED_EDGE('',*,*,#47820,.T.);
#63561=ORIENTED_EDGE('',*,*,#47821,.T.);
#63562=ORIENTED_EDGE('',*,*,#47822,.T.);
#63563=ORIENTED_EDGE('',*,*,#47823,.T.);
#63564=ORIENTED_EDGE('',*,*,#47824,.T.);
#63565=ORIENTED_EDGE('',*,*,#47825,.T.);
#63566=ORIENTED_EDGE('',*,*,#47826,.F.);
#63567=ORIENTED_EDGE('',*,*,#47827,.F.);
#63568=ORIENTED_EDGE('',*,*,#47828,.F.);
#63569=ORIENTED_EDGE('',*,*,#47829,.T.);
#63570=ORIENTED_EDGE('',*,*,#47827,.T.);
#63571=ORIENTED_EDGE('',*,*,#47830,.T.);
#63572=ORIENTED_EDGE('',*,*,#47831,.T.);
#63573=ORIENTED_EDGE('',*,*,#47832,.T.);
#63574=ORIENTED_EDGE('',*,*,#46332,.F.);
#63575=ORIENTED_EDGE('',*,*,#47833,.T.);
#63576=ORIENTED_EDGE('',*,*,#47811,.F.);
#63577=ORIENTED_EDGE('',*,*,#47834,.T.);
#63578=ORIENTED_EDGE('',*,*,#47831,.F.);
#63579=ORIENTED_EDGE('',*,*,#47835,.T.);
#63580=ORIENTED_EDGE('',*,*,#46040,.F.);
#63581=ORIENTED_EDGE('',*,*,#47836,.T.);
#63582=ORIENTED_EDGE('',*,*,#47822,.F.);
#63583=ORIENTED_EDGE('',*,*,#47837,.T.);
#63584=ORIENTED_EDGE('',*,*,#47824,.F.);
#63585=ORIENTED_EDGE('',*,*,#47838,.T.);
#63586=ORIENTED_EDGE('',*,*,#47818,.F.);
#63587=ORIENTED_EDGE('',*,*,#47839,.T.);
#63588=ORIENTED_EDGE('',*,*,#47820,.F.);
#63589=ORIENTED_EDGE('',*,*,#47840,.T.);
#63590=ORIENTED_EDGE('',*,*,#47841,.T.);
#63591=ORIENTED_EDGE('',*,*,#47842,.T.);
#63592=ORIENTED_EDGE('',*,*,#47843,.F.);
#63593=ORIENTED_EDGE('',*,*,#47844,.F.);
#63594=ORIENTED_EDGE('',*,*,#47845,.F.);
#63595=ORIENTED_EDGE('',*,*,#47846,.T.);
#63596=ORIENTED_EDGE('',*,*,#47844,.T.);
#63597=ORIENTED_EDGE('',*,*,#47847,.T.);
#63598=ORIENTED_EDGE('',*,*,#47848,.T.);
#63599=ORIENTED_EDGE('',*,*,#47849,.T.);
#63600=ORIENTED_EDGE('',*,*,#47850,.T.);
#63601=ORIENTED_EDGE('',*,*,#47851,.T.);
#63602=ORIENTED_EDGE('',*,*,#47852,.T.);
#63603=ORIENTED_EDGE('',*,*,#47853,.T.);
#63604=ORIENTED_EDGE('',*,*,#47854,.T.);
#63605=ORIENTED_EDGE('',*,*,#47855,.T.);
#63606=ORIENTED_EDGE('',*,*,#47856,.F.);
#63607=ORIENTED_EDGE('',*,*,#47857,.F.);
#63608=ORIENTED_EDGE('',*,*,#47858,.F.);
#63609=ORIENTED_EDGE('',*,*,#47859,.T.);
#63610=ORIENTED_EDGE('',*,*,#47857,.T.);
#63611=ORIENTED_EDGE('',*,*,#47860,.T.);
#63612=ORIENTED_EDGE('',*,*,#47861,.T.);
#63613=ORIENTED_EDGE('',*,*,#47862,.T.);
#63614=ORIENTED_EDGE('',*,*,#46338,.F.);
#63615=ORIENTED_EDGE('',*,*,#47863,.T.);
#63616=ORIENTED_EDGE('',*,*,#47841,.F.);
#63617=ORIENTED_EDGE('',*,*,#47864,.T.);
#63618=ORIENTED_EDGE('',*,*,#47861,.F.);
#63619=ORIENTED_EDGE('',*,*,#47865,.T.);
#63620=ORIENTED_EDGE('',*,*,#46034,.F.);
#63621=ORIENTED_EDGE('',*,*,#47866,.T.);
#63622=ORIENTED_EDGE('',*,*,#47852,.F.);
#63623=ORIENTED_EDGE('',*,*,#47867,.T.);
#63624=ORIENTED_EDGE('',*,*,#47854,.F.);
#63625=ORIENTED_EDGE('',*,*,#47868,.T.);
#63626=ORIENTED_EDGE('',*,*,#47848,.F.);
#63627=ORIENTED_EDGE('',*,*,#47869,.T.);
#63628=ORIENTED_EDGE('',*,*,#47850,.F.);
#63629=ORIENTED_EDGE('',*,*,#47870,.T.);
#63630=ORIENTED_EDGE('',*,*,#47871,.T.);
#63631=ORIENTED_EDGE('',*,*,#47872,.T.);
#63632=ORIENTED_EDGE('',*,*,#47873,.F.);
#63633=ORIENTED_EDGE('',*,*,#47874,.F.);
#63634=ORIENTED_EDGE('',*,*,#47875,.F.);
#63635=ORIENTED_EDGE('',*,*,#47876,.T.);
#63636=ORIENTED_EDGE('',*,*,#47874,.T.);
#63637=ORIENTED_EDGE('',*,*,#47877,.T.);
#63638=ORIENTED_EDGE('',*,*,#47878,.T.);
#63639=ORIENTED_EDGE('',*,*,#47879,.T.);
#63640=ORIENTED_EDGE('',*,*,#47880,.T.);
#63641=ORIENTED_EDGE('',*,*,#47881,.T.);
#63642=ORIENTED_EDGE('',*,*,#47882,.T.);
#63643=ORIENTED_EDGE('',*,*,#47883,.T.);
#63644=ORIENTED_EDGE('',*,*,#47884,.T.);
#63645=ORIENTED_EDGE('',*,*,#47885,.T.);
#63646=ORIENTED_EDGE('',*,*,#47886,.F.);
#63647=ORIENTED_EDGE('',*,*,#47887,.F.);
#63648=ORIENTED_EDGE('',*,*,#47888,.F.);
#63649=ORIENTED_EDGE('',*,*,#47889,.T.);
#63650=ORIENTED_EDGE('',*,*,#47887,.T.);
#63651=ORIENTED_EDGE('',*,*,#47890,.T.);
#63652=ORIENTED_EDGE('',*,*,#47891,.T.);
#63653=ORIENTED_EDGE('',*,*,#47892,.T.);
#63654=ORIENTED_EDGE('',*,*,#46344,.F.);
#63655=ORIENTED_EDGE('',*,*,#47893,.T.);
#63656=ORIENTED_EDGE('',*,*,#47871,.F.);
#63657=ORIENTED_EDGE('',*,*,#47894,.T.);
#63658=ORIENTED_EDGE('',*,*,#47891,.F.);
#63659=ORIENTED_EDGE('',*,*,#47895,.T.);
#63660=ORIENTED_EDGE('',*,*,#46028,.F.);
#63661=ORIENTED_EDGE('',*,*,#47896,.T.);
#63662=ORIENTED_EDGE('',*,*,#47882,.F.);
#63663=ORIENTED_EDGE('',*,*,#47897,.T.);
#63664=ORIENTED_EDGE('',*,*,#47884,.F.);
#63665=ORIENTED_EDGE('',*,*,#47898,.T.);
#63666=ORIENTED_EDGE('',*,*,#47878,.F.);
#63667=ORIENTED_EDGE('',*,*,#47899,.T.);
#63668=ORIENTED_EDGE('',*,*,#47880,.F.);
#63669=ORIENTED_EDGE('',*,*,#47900,.T.);
#63670=ORIENTED_EDGE('',*,*,#47901,.T.);
#63671=ORIENTED_EDGE('',*,*,#47902,.T.);
#63672=ORIENTED_EDGE('',*,*,#47903,.F.);
#63673=ORIENTED_EDGE('',*,*,#47904,.F.);
#63674=ORIENTED_EDGE('',*,*,#47905,.F.);
#63675=ORIENTED_EDGE('',*,*,#47906,.T.);
#63676=ORIENTED_EDGE('',*,*,#47904,.T.);
#63677=ORIENTED_EDGE('',*,*,#47907,.T.);
#63678=ORIENTED_EDGE('',*,*,#47908,.T.);
#63679=ORIENTED_EDGE('',*,*,#47909,.T.);
#63680=ORIENTED_EDGE('',*,*,#47910,.T.);
#63681=ORIENTED_EDGE('',*,*,#47911,.T.);
#63682=ORIENTED_EDGE('',*,*,#47912,.T.);
#63683=ORIENTED_EDGE('',*,*,#47913,.T.);
#63684=ORIENTED_EDGE('',*,*,#47914,.T.);
#63685=ORIENTED_EDGE('',*,*,#47915,.T.);
#63686=ORIENTED_EDGE('',*,*,#47916,.F.);
#63687=ORIENTED_EDGE('',*,*,#47917,.F.);
#63688=ORIENTED_EDGE('',*,*,#47918,.F.);
#63689=ORIENTED_EDGE('',*,*,#47919,.T.);
#63690=ORIENTED_EDGE('',*,*,#47917,.T.);
#63691=ORIENTED_EDGE('',*,*,#47920,.T.);
#63692=ORIENTED_EDGE('',*,*,#47921,.T.);
#63693=ORIENTED_EDGE('',*,*,#47922,.T.);
#63694=ORIENTED_EDGE('',*,*,#46350,.F.);
#63695=ORIENTED_EDGE('',*,*,#47923,.T.);
#63696=ORIENTED_EDGE('',*,*,#47901,.F.);
#63697=ORIENTED_EDGE('',*,*,#47924,.T.);
#63698=ORIENTED_EDGE('',*,*,#47921,.F.);
#63699=ORIENTED_EDGE('',*,*,#47925,.T.);
#63700=ORIENTED_EDGE('',*,*,#46022,.F.);
#63701=ORIENTED_EDGE('',*,*,#47926,.T.);
#63702=ORIENTED_EDGE('',*,*,#47912,.F.);
#63703=ORIENTED_EDGE('',*,*,#47927,.T.);
#63704=ORIENTED_EDGE('',*,*,#47914,.F.);
#63705=ORIENTED_EDGE('',*,*,#47928,.T.);
#63706=ORIENTED_EDGE('',*,*,#47908,.F.);
#63707=ORIENTED_EDGE('',*,*,#47929,.T.);
#63708=ORIENTED_EDGE('',*,*,#47910,.F.);
#63709=ORIENTED_EDGE('',*,*,#47930,.T.);
#63710=ORIENTED_EDGE('',*,*,#47931,.T.);
#63711=ORIENTED_EDGE('',*,*,#47932,.T.);
#63712=ORIENTED_EDGE('',*,*,#47933,.F.);
#63713=ORIENTED_EDGE('',*,*,#47934,.F.);
#63714=ORIENTED_EDGE('',*,*,#47935,.F.);
#63715=ORIENTED_EDGE('',*,*,#47936,.T.);
#63716=ORIENTED_EDGE('',*,*,#47934,.T.);
#63717=ORIENTED_EDGE('',*,*,#47937,.T.);
#63718=ORIENTED_EDGE('',*,*,#47938,.T.);
#63719=ORIENTED_EDGE('',*,*,#47939,.T.);
#63720=ORIENTED_EDGE('',*,*,#47940,.T.);
#63721=ORIENTED_EDGE('',*,*,#47941,.T.);
#63722=ORIENTED_EDGE('',*,*,#47942,.T.);
#63723=ORIENTED_EDGE('',*,*,#47943,.T.);
#63724=ORIENTED_EDGE('',*,*,#47944,.T.);
#63725=ORIENTED_EDGE('',*,*,#47945,.T.);
#63726=ORIENTED_EDGE('',*,*,#47946,.F.);
#63727=ORIENTED_EDGE('',*,*,#47947,.F.);
#63728=ORIENTED_EDGE('',*,*,#47948,.F.);
#63729=ORIENTED_EDGE('',*,*,#47949,.T.);
#63730=ORIENTED_EDGE('',*,*,#47947,.T.);
#63731=ORIENTED_EDGE('',*,*,#47950,.T.);
#63732=ORIENTED_EDGE('',*,*,#47951,.T.);
#63733=ORIENTED_EDGE('',*,*,#47952,.T.);
#63734=ORIENTED_EDGE('',*,*,#46356,.F.);
#63735=ORIENTED_EDGE('',*,*,#47953,.T.);
#63736=ORIENTED_EDGE('',*,*,#47931,.F.);
#63737=ORIENTED_EDGE('',*,*,#47954,.T.);
#63738=ORIENTED_EDGE('',*,*,#47951,.F.);
#63739=ORIENTED_EDGE('',*,*,#47955,.T.);
#63740=ORIENTED_EDGE('',*,*,#46016,.F.);
#63741=ORIENTED_EDGE('',*,*,#47956,.T.);
#63742=ORIENTED_EDGE('',*,*,#47942,.F.);
#63743=ORIENTED_EDGE('',*,*,#47957,.T.);
#63744=ORIENTED_EDGE('',*,*,#47944,.F.);
#63745=ORIENTED_EDGE('',*,*,#47958,.T.);
#63746=ORIENTED_EDGE('',*,*,#47938,.F.);
#63747=ORIENTED_EDGE('',*,*,#47959,.T.);
#63748=ORIENTED_EDGE('',*,*,#47940,.F.);
#63749=ORIENTED_EDGE('',*,*,#47960,.T.);
#63750=ORIENTED_EDGE('',*,*,#47961,.T.);
#63751=ORIENTED_EDGE('',*,*,#47962,.T.);
#63752=ORIENTED_EDGE('',*,*,#47963,.F.);
#63753=ORIENTED_EDGE('',*,*,#47964,.F.);
#63754=ORIENTED_EDGE('',*,*,#47965,.F.);
#63755=ORIENTED_EDGE('',*,*,#47966,.T.);
#63756=ORIENTED_EDGE('',*,*,#47964,.T.);
#63757=ORIENTED_EDGE('',*,*,#47967,.T.);
#63758=ORIENTED_EDGE('',*,*,#47968,.T.);
#63759=ORIENTED_EDGE('',*,*,#47969,.T.);
#63760=ORIENTED_EDGE('',*,*,#47970,.T.);
#63761=ORIENTED_EDGE('',*,*,#47971,.T.);
#63762=ORIENTED_EDGE('',*,*,#47972,.T.);
#63763=ORIENTED_EDGE('',*,*,#47973,.T.);
#63764=ORIENTED_EDGE('',*,*,#47974,.T.);
#63765=ORIENTED_EDGE('',*,*,#47975,.T.);
#63766=ORIENTED_EDGE('',*,*,#47976,.F.);
#63767=ORIENTED_EDGE('',*,*,#47977,.F.);
#63768=ORIENTED_EDGE('',*,*,#47978,.F.);
#63769=ORIENTED_EDGE('',*,*,#47979,.T.);
#63770=ORIENTED_EDGE('',*,*,#47977,.T.);
#63771=ORIENTED_EDGE('',*,*,#47980,.T.);
#63772=ORIENTED_EDGE('',*,*,#47981,.T.);
#63773=ORIENTED_EDGE('',*,*,#47982,.T.);
#63774=ORIENTED_EDGE('',*,*,#46362,.F.);
#63775=ORIENTED_EDGE('',*,*,#47983,.T.);
#63776=ORIENTED_EDGE('',*,*,#47961,.F.);
#63777=ORIENTED_EDGE('',*,*,#47984,.T.);
#63778=ORIENTED_EDGE('',*,*,#47981,.F.);
#63779=ORIENTED_EDGE('',*,*,#47985,.T.);
#63780=ORIENTED_EDGE('',*,*,#46010,.F.);
#63781=ORIENTED_EDGE('',*,*,#47986,.T.);
#63782=ORIENTED_EDGE('',*,*,#47972,.F.);
#63783=ORIENTED_EDGE('',*,*,#47987,.T.);
#63784=ORIENTED_EDGE('',*,*,#47974,.F.);
#63785=ORIENTED_EDGE('',*,*,#47988,.T.);
#63786=ORIENTED_EDGE('',*,*,#47968,.F.);
#63787=ORIENTED_EDGE('',*,*,#47989,.T.);
#63788=ORIENTED_EDGE('',*,*,#47970,.F.);
#63789=ORIENTED_EDGE('',*,*,#47990,.T.);
#63790=ORIENTED_EDGE('',*,*,#47991,.T.);
#63791=ORIENTED_EDGE('',*,*,#47992,.T.);
#63792=ORIENTED_EDGE('',*,*,#47993,.F.);
#63793=ORIENTED_EDGE('',*,*,#47994,.F.);
#63794=ORIENTED_EDGE('',*,*,#47995,.F.);
#63795=ORIENTED_EDGE('',*,*,#47996,.T.);
#63796=ORIENTED_EDGE('',*,*,#47994,.T.);
#63797=ORIENTED_EDGE('',*,*,#47997,.T.);
#63798=ORIENTED_EDGE('',*,*,#47998,.T.);
#63799=ORIENTED_EDGE('',*,*,#47999,.T.);
#63800=ORIENTED_EDGE('',*,*,#48000,.T.);
#63801=ORIENTED_EDGE('',*,*,#48001,.T.);
#63802=ORIENTED_EDGE('',*,*,#48002,.T.);
#63803=ORIENTED_EDGE('',*,*,#48003,.T.);
#63804=ORIENTED_EDGE('',*,*,#48004,.T.);
#63805=ORIENTED_EDGE('',*,*,#48005,.T.);
#63806=ORIENTED_EDGE('',*,*,#48006,.F.);
#63807=ORIENTED_EDGE('',*,*,#48007,.F.);
#63808=ORIENTED_EDGE('',*,*,#48008,.F.);
#63809=ORIENTED_EDGE('',*,*,#48009,.T.);
#63810=ORIENTED_EDGE('',*,*,#48007,.T.);
#63811=ORIENTED_EDGE('',*,*,#48010,.T.);
#63812=ORIENTED_EDGE('',*,*,#48011,.T.);
#63813=ORIENTED_EDGE('',*,*,#48012,.T.);
#63814=ORIENTED_EDGE('',*,*,#46368,.F.);
#63815=ORIENTED_EDGE('',*,*,#48013,.T.);
#63816=ORIENTED_EDGE('',*,*,#47991,.F.);
#63817=ORIENTED_EDGE('',*,*,#48014,.T.);
#63818=ORIENTED_EDGE('',*,*,#48011,.F.);
#63819=ORIENTED_EDGE('',*,*,#48015,.T.);
#63820=ORIENTED_EDGE('',*,*,#46004,.F.);
#63821=ORIENTED_EDGE('',*,*,#48016,.T.);
#63822=ORIENTED_EDGE('',*,*,#48002,.F.);
#63823=ORIENTED_EDGE('',*,*,#48017,.T.);
#63824=ORIENTED_EDGE('',*,*,#48004,.F.);
#63825=ORIENTED_EDGE('',*,*,#48018,.T.);
#63826=ORIENTED_EDGE('',*,*,#47998,.F.);
#63827=ORIENTED_EDGE('',*,*,#48019,.T.);
#63828=ORIENTED_EDGE('',*,*,#48000,.F.);
#63829=ORIENTED_EDGE('',*,*,#48020,.T.);
#63830=ORIENTED_EDGE('',*,*,#48021,.T.);
#63831=ORIENTED_EDGE('',*,*,#48022,.T.);
#63832=ORIENTED_EDGE('',*,*,#48023,.F.);
#63833=ORIENTED_EDGE('',*,*,#48024,.F.);
#63834=ORIENTED_EDGE('',*,*,#48025,.F.);
#63835=ORIENTED_EDGE('',*,*,#48026,.T.);
#63836=ORIENTED_EDGE('',*,*,#48024,.T.);
#63837=ORIENTED_EDGE('',*,*,#48027,.T.);
#63838=ORIENTED_EDGE('',*,*,#48028,.T.);
#63839=ORIENTED_EDGE('',*,*,#48029,.T.);
#63840=ORIENTED_EDGE('',*,*,#48030,.T.);
#63841=ORIENTED_EDGE('',*,*,#48031,.T.);
#63842=ORIENTED_EDGE('',*,*,#48032,.T.);
#63843=ORIENTED_EDGE('',*,*,#48033,.T.);
#63844=ORIENTED_EDGE('',*,*,#48034,.T.);
#63845=ORIENTED_EDGE('',*,*,#48035,.T.);
#63846=ORIENTED_EDGE('',*,*,#48036,.F.);
#63847=ORIENTED_EDGE('',*,*,#48037,.F.);
#63848=ORIENTED_EDGE('',*,*,#48038,.F.);
#63849=ORIENTED_EDGE('',*,*,#48039,.T.);
#63850=ORIENTED_EDGE('',*,*,#48037,.T.);
#63851=ORIENTED_EDGE('',*,*,#48040,.T.);
#63852=ORIENTED_EDGE('',*,*,#48041,.T.);
#63853=ORIENTED_EDGE('',*,*,#48042,.T.);
#63854=ORIENTED_EDGE('',*,*,#46374,.F.);
#63855=ORIENTED_EDGE('',*,*,#48043,.T.);
#63856=ORIENTED_EDGE('',*,*,#48021,.F.);
#63857=ORIENTED_EDGE('',*,*,#48044,.T.);
#63858=ORIENTED_EDGE('',*,*,#48041,.F.);
#63859=ORIENTED_EDGE('',*,*,#48045,.T.);
#63860=ORIENTED_EDGE('',*,*,#45998,.F.);
#63861=ORIENTED_EDGE('',*,*,#48046,.T.);
#63862=ORIENTED_EDGE('',*,*,#48032,.F.);
#63863=ORIENTED_EDGE('',*,*,#48047,.T.);
#63864=ORIENTED_EDGE('',*,*,#48034,.F.);
#63865=ORIENTED_EDGE('',*,*,#48048,.T.);
#63866=ORIENTED_EDGE('',*,*,#48028,.F.);
#63867=ORIENTED_EDGE('',*,*,#48049,.T.);
#63868=ORIENTED_EDGE('',*,*,#48030,.F.);
#63869=ORIENTED_EDGE('',*,*,#48050,.T.);
#63870=ORIENTED_EDGE('',*,*,#48051,.T.);
#63871=ORIENTED_EDGE('',*,*,#48052,.T.);
#63872=ORIENTED_EDGE('',*,*,#48053,.F.);
#63873=ORIENTED_EDGE('',*,*,#48054,.F.);
#63874=ORIENTED_EDGE('',*,*,#48055,.F.);
#63875=ORIENTED_EDGE('',*,*,#48056,.T.);
#63876=ORIENTED_EDGE('',*,*,#48054,.T.);
#63877=ORIENTED_EDGE('',*,*,#48057,.T.);
#63878=ORIENTED_EDGE('',*,*,#48058,.T.);
#63879=ORIENTED_EDGE('',*,*,#48059,.T.);
#63880=ORIENTED_EDGE('',*,*,#48060,.T.);
#63881=ORIENTED_EDGE('',*,*,#48061,.T.);
#63882=ORIENTED_EDGE('',*,*,#48062,.T.);
#63883=ORIENTED_EDGE('',*,*,#48063,.T.);
#63884=ORIENTED_EDGE('',*,*,#48064,.T.);
#63885=ORIENTED_EDGE('',*,*,#48065,.T.);
#63886=ORIENTED_EDGE('',*,*,#48066,.F.);
#63887=ORIENTED_EDGE('',*,*,#48067,.F.);
#63888=ORIENTED_EDGE('',*,*,#48068,.F.);
#63889=ORIENTED_EDGE('',*,*,#48069,.T.);
#63890=ORIENTED_EDGE('',*,*,#48067,.T.);
#63891=ORIENTED_EDGE('',*,*,#48070,.T.);
#63892=ORIENTED_EDGE('',*,*,#48071,.T.);
#63893=ORIENTED_EDGE('',*,*,#48072,.T.);
#63894=ORIENTED_EDGE('',*,*,#46380,.F.);
#63895=ORIENTED_EDGE('',*,*,#48073,.T.);
#63896=ORIENTED_EDGE('',*,*,#48051,.F.);
#63897=ORIENTED_EDGE('',*,*,#48074,.T.);
#63898=ORIENTED_EDGE('',*,*,#48071,.F.);
#63899=ORIENTED_EDGE('',*,*,#48075,.T.);
#63900=ORIENTED_EDGE('',*,*,#45992,.F.);
#63901=ORIENTED_EDGE('',*,*,#48076,.T.);
#63902=ORIENTED_EDGE('',*,*,#48062,.F.);
#63903=ORIENTED_EDGE('',*,*,#48077,.T.);
#63904=ORIENTED_EDGE('',*,*,#48064,.F.);
#63905=ORIENTED_EDGE('',*,*,#48078,.T.);
#63906=ORIENTED_EDGE('',*,*,#48058,.F.);
#63907=ORIENTED_EDGE('',*,*,#48079,.T.);
#63908=ORIENTED_EDGE('',*,*,#48060,.F.);
#63909=ORIENTED_EDGE('',*,*,#48080,.T.);
#63910=ORIENTED_EDGE('',*,*,#48081,.T.);
#63911=ORIENTED_EDGE('',*,*,#48082,.T.);
#63912=ORIENTED_EDGE('',*,*,#48083,.F.);
#63913=ORIENTED_EDGE('',*,*,#48084,.F.);
#63914=ORIENTED_EDGE('',*,*,#48085,.F.);
#63915=ORIENTED_EDGE('',*,*,#48086,.T.);
#63916=ORIENTED_EDGE('',*,*,#48084,.T.);
#63917=ORIENTED_EDGE('',*,*,#48087,.T.);
#63918=ORIENTED_EDGE('',*,*,#48088,.T.);
#63919=ORIENTED_EDGE('',*,*,#48089,.T.);
#63920=ORIENTED_EDGE('',*,*,#48090,.T.);
#63921=ORIENTED_EDGE('',*,*,#48091,.T.);
#63922=ORIENTED_EDGE('',*,*,#48092,.T.);
#63923=ORIENTED_EDGE('',*,*,#48093,.T.);
#63924=ORIENTED_EDGE('',*,*,#48094,.T.);
#63925=ORIENTED_EDGE('',*,*,#48095,.T.);
#63926=ORIENTED_EDGE('',*,*,#48096,.F.);
#63927=ORIENTED_EDGE('',*,*,#48097,.F.);
#63928=ORIENTED_EDGE('',*,*,#48098,.F.);
#63929=ORIENTED_EDGE('',*,*,#48099,.T.);
#63930=ORIENTED_EDGE('',*,*,#48097,.T.);
#63931=ORIENTED_EDGE('',*,*,#48100,.T.);
#63932=ORIENTED_EDGE('',*,*,#48101,.T.);
#63933=ORIENTED_EDGE('',*,*,#48102,.T.);
#63934=ORIENTED_EDGE('',*,*,#46386,.F.);
#63935=ORIENTED_EDGE('',*,*,#48103,.T.);
#63936=ORIENTED_EDGE('',*,*,#48081,.F.);
#63937=ORIENTED_EDGE('',*,*,#48104,.T.);
#63938=ORIENTED_EDGE('',*,*,#48101,.F.);
#63939=ORIENTED_EDGE('',*,*,#48105,.T.);
#63940=ORIENTED_EDGE('',*,*,#45986,.F.);
#63941=ORIENTED_EDGE('',*,*,#48106,.T.);
#63942=ORIENTED_EDGE('',*,*,#48092,.F.);
#63943=ORIENTED_EDGE('',*,*,#48107,.T.);
#63944=ORIENTED_EDGE('',*,*,#48094,.F.);
#63945=ORIENTED_EDGE('',*,*,#48108,.T.);
#63946=ORIENTED_EDGE('',*,*,#48088,.F.);
#63947=ORIENTED_EDGE('',*,*,#48109,.T.);
#63948=ORIENTED_EDGE('',*,*,#48090,.F.);
#63949=ORIENTED_EDGE('',*,*,#48110,.T.);
#63950=ORIENTED_EDGE('',*,*,#48111,.T.);
#63951=ORIENTED_EDGE('',*,*,#48112,.T.);
#63952=ORIENTED_EDGE('',*,*,#48113,.F.);
#63953=ORIENTED_EDGE('',*,*,#48114,.F.);
#63954=ORIENTED_EDGE('',*,*,#48115,.F.);
#63955=ORIENTED_EDGE('',*,*,#48116,.T.);
#63956=ORIENTED_EDGE('',*,*,#48114,.T.);
#63957=ORIENTED_EDGE('',*,*,#48117,.T.);
#63958=ORIENTED_EDGE('',*,*,#48118,.T.);
#63959=ORIENTED_EDGE('',*,*,#48119,.T.);
#63960=ORIENTED_EDGE('',*,*,#48120,.T.);
#63961=ORIENTED_EDGE('',*,*,#48121,.T.);
#63962=ORIENTED_EDGE('',*,*,#48122,.T.);
#63963=ORIENTED_EDGE('',*,*,#48123,.T.);
#63964=ORIENTED_EDGE('',*,*,#48124,.T.);
#63965=ORIENTED_EDGE('',*,*,#48125,.T.);
#63966=ORIENTED_EDGE('',*,*,#48126,.F.);
#63967=ORIENTED_EDGE('',*,*,#48127,.F.);
#63968=ORIENTED_EDGE('',*,*,#48128,.F.);
#63969=ORIENTED_EDGE('',*,*,#48129,.T.);
#63970=ORIENTED_EDGE('',*,*,#48127,.T.);
#63971=ORIENTED_EDGE('',*,*,#48130,.T.);
#63972=ORIENTED_EDGE('',*,*,#48131,.T.);
#63973=ORIENTED_EDGE('',*,*,#48132,.T.);
#63974=ORIENTED_EDGE('',*,*,#46392,.F.);
#63975=ORIENTED_EDGE('',*,*,#48133,.T.);
#63976=ORIENTED_EDGE('',*,*,#48111,.F.);
#63977=ORIENTED_EDGE('',*,*,#48134,.T.);
#63978=ORIENTED_EDGE('',*,*,#48131,.F.);
#63979=ORIENTED_EDGE('',*,*,#48135,.T.);
#63980=ORIENTED_EDGE('',*,*,#45980,.F.);
#63981=ORIENTED_EDGE('',*,*,#48136,.T.);
#63982=ORIENTED_EDGE('',*,*,#48122,.F.);
#63983=ORIENTED_EDGE('',*,*,#48137,.T.);
#63984=ORIENTED_EDGE('',*,*,#48124,.F.);
#63985=ORIENTED_EDGE('',*,*,#48138,.T.);
#63986=ORIENTED_EDGE('',*,*,#48118,.F.);
#63987=ORIENTED_EDGE('',*,*,#48139,.T.);
#63988=ORIENTED_EDGE('',*,*,#48120,.F.);
#63989=ORIENTED_EDGE('',*,*,#48140,.T.);
#63990=ORIENTED_EDGE('',*,*,#48141,.T.);
#63991=ORIENTED_EDGE('',*,*,#48142,.T.);
#63992=ORIENTED_EDGE('',*,*,#48143,.F.);
#63993=ORIENTED_EDGE('',*,*,#48144,.F.);
#63994=ORIENTED_EDGE('',*,*,#48145,.F.);
#63995=ORIENTED_EDGE('',*,*,#48146,.T.);
#63996=ORIENTED_EDGE('',*,*,#48144,.T.);
#63997=ORIENTED_EDGE('',*,*,#48147,.T.);
#63998=ORIENTED_EDGE('',*,*,#48148,.T.);
#63999=ORIENTED_EDGE('',*,*,#48149,.T.);
#64000=ORIENTED_EDGE('',*,*,#48150,.T.);
#64001=ORIENTED_EDGE('',*,*,#48151,.T.);
#64002=ORIENTED_EDGE('',*,*,#48152,.T.);
#64003=ORIENTED_EDGE('',*,*,#48153,.T.);
#64004=ORIENTED_EDGE('',*,*,#48154,.T.);
#64005=ORIENTED_EDGE('',*,*,#48155,.T.);
#64006=ORIENTED_EDGE('',*,*,#48156,.F.);
#64007=ORIENTED_EDGE('',*,*,#48157,.F.);
#64008=ORIENTED_EDGE('',*,*,#48158,.F.);
#64009=ORIENTED_EDGE('',*,*,#48159,.T.);
#64010=ORIENTED_EDGE('',*,*,#48157,.T.);
#64011=ORIENTED_EDGE('',*,*,#48160,.T.);
#64012=ORIENTED_EDGE('',*,*,#48161,.T.);
#64013=ORIENTED_EDGE('',*,*,#48162,.T.);
#64014=ORIENTED_EDGE('',*,*,#46398,.F.);
#64015=ORIENTED_EDGE('',*,*,#48163,.T.);
#64016=ORIENTED_EDGE('',*,*,#48141,.F.);
#64017=ORIENTED_EDGE('',*,*,#48164,.T.);
#64018=ORIENTED_EDGE('',*,*,#48161,.F.);
#64019=ORIENTED_EDGE('',*,*,#48165,.T.);
#64020=ORIENTED_EDGE('',*,*,#45974,.F.);
#64021=ORIENTED_EDGE('',*,*,#48166,.T.);
#64022=ORIENTED_EDGE('',*,*,#48152,.F.);
#64023=ORIENTED_EDGE('',*,*,#48167,.T.);
#64024=ORIENTED_EDGE('',*,*,#48154,.F.);
#64025=ORIENTED_EDGE('',*,*,#48168,.T.);
#64026=ORIENTED_EDGE('',*,*,#48148,.F.);
#64027=ORIENTED_EDGE('',*,*,#48169,.T.);
#64028=ORIENTED_EDGE('',*,*,#48150,.F.);
#64029=ORIENTED_EDGE('',*,*,#48170,.T.);
#64030=ORIENTED_EDGE('',*,*,#48171,.T.);
#64031=ORIENTED_EDGE('',*,*,#48172,.T.);
#64032=ORIENTED_EDGE('',*,*,#48173,.F.);
#64033=ORIENTED_EDGE('',*,*,#48174,.F.);
#64034=ORIENTED_EDGE('',*,*,#48175,.F.);
#64035=ORIENTED_EDGE('',*,*,#48176,.T.);
#64036=ORIENTED_EDGE('',*,*,#48174,.T.);
#64037=ORIENTED_EDGE('',*,*,#48177,.T.);
#64038=ORIENTED_EDGE('',*,*,#48178,.T.);
#64039=ORIENTED_EDGE('',*,*,#48179,.T.);
#64040=ORIENTED_EDGE('',*,*,#48180,.T.);
#64041=ORIENTED_EDGE('',*,*,#48181,.T.);
#64042=ORIENTED_EDGE('',*,*,#48182,.T.);
#64043=ORIENTED_EDGE('',*,*,#48183,.T.);
#64044=ORIENTED_EDGE('',*,*,#48184,.T.);
#64045=ORIENTED_EDGE('',*,*,#48185,.T.);
#64046=ORIENTED_EDGE('',*,*,#48186,.F.);
#64047=ORIENTED_EDGE('',*,*,#48187,.F.);
#64048=ORIENTED_EDGE('',*,*,#48188,.F.);
#64049=ORIENTED_EDGE('',*,*,#48189,.T.);
#64050=ORIENTED_EDGE('',*,*,#48187,.T.);
#64051=ORIENTED_EDGE('',*,*,#48190,.T.);
#64052=ORIENTED_EDGE('',*,*,#48191,.T.);
#64053=ORIENTED_EDGE('',*,*,#48192,.T.);
#64054=ORIENTED_EDGE('',*,*,#46404,.F.);
#64055=ORIENTED_EDGE('',*,*,#48193,.T.);
#64056=ORIENTED_EDGE('',*,*,#48171,.F.);
#64057=ORIENTED_EDGE('',*,*,#48194,.T.);
#64058=ORIENTED_EDGE('',*,*,#48191,.F.);
#64059=ORIENTED_EDGE('',*,*,#48195,.T.);
#64060=ORIENTED_EDGE('',*,*,#45968,.F.);
#64061=ORIENTED_EDGE('',*,*,#48196,.T.);
#64062=ORIENTED_EDGE('',*,*,#48182,.F.);
#64063=ORIENTED_EDGE('',*,*,#48197,.T.);
#64064=ORIENTED_EDGE('',*,*,#48184,.F.);
#64065=ORIENTED_EDGE('',*,*,#48198,.T.);
#64066=ORIENTED_EDGE('',*,*,#48178,.F.);
#64067=ORIENTED_EDGE('',*,*,#48199,.T.);
#64068=ORIENTED_EDGE('',*,*,#48180,.F.);
#64069=ORIENTED_EDGE('',*,*,#48200,.T.);
#64070=ORIENTED_EDGE('',*,*,#48201,.T.);
#64071=ORIENTED_EDGE('',*,*,#48202,.T.);
#64072=ORIENTED_EDGE('',*,*,#48203,.F.);
#64073=ORIENTED_EDGE('',*,*,#48204,.F.);
#64074=ORIENTED_EDGE('',*,*,#48205,.F.);
#64075=ORIENTED_EDGE('',*,*,#48206,.T.);
#64076=ORIENTED_EDGE('',*,*,#48204,.T.);
#64077=ORIENTED_EDGE('',*,*,#48207,.T.);
#64078=ORIENTED_EDGE('',*,*,#48208,.T.);
#64079=ORIENTED_EDGE('',*,*,#48209,.T.);
#64080=ORIENTED_EDGE('',*,*,#48210,.T.);
#64081=ORIENTED_EDGE('',*,*,#48211,.T.);
#64082=ORIENTED_EDGE('',*,*,#48212,.T.);
#64083=ORIENTED_EDGE('',*,*,#48213,.T.);
#64084=ORIENTED_EDGE('',*,*,#48214,.T.);
#64085=ORIENTED_EDGE('',*,*,#48215,.T.);
#64086=ORIENTED_EDGE('',*,*,#48216,.F.);
#64087=ORIENTED_EDGE('',*,*,#48217,.F.);
#64088=ORIENTED_EDGE('',*,*,#48218,.F.);
#64089=ORIENTED_EDGE('',*,*,#48219,.T.);
#64090=ORIENTED_EDGE('',*,*,#48217,.T.);
#64091=ORIENTED_EDGE('',*,*,#48220,.T.);
#64092=ORIENTED_EDGE('',*,*,#48221,.T.);
#64093=ORIENTED_EDGE('',*,*,#48222,.T.);
#64094=ORIENTED_EDGE('',*,*,#46410,.F.);
#64095=ORIENTED_EDGE('',*,*,#48223,.T.);
#64096=ORIENTED_EDGE('',*,*,#48201,.F.);
#64097=ORIENTED_EDGE('',*,*,#48224,.T.);
#64098=ORIENTED_EDGE('',*,*,#48221,.F.);
#64099=ORIENTED_EDGE('',*,*,#48225,.T.);
#64100=ORIENTED_EDGE('',*,*,#45962,.F.);
#64101=ORIENTED_EDGE('',*,*,#48226,.T.);
#64102=ORIENTED_EDGE('',*,*,#48212,.F.);
#64103=ORIENTED_EDGE('',*,*,#48227,.T.);
#64104=ORIENTED_EDGE('',*,*,#48214,.F.);
#64105=ORIENTED_EDGE('',*,*,#48228,.T.);
#64106=ORIENTED_EDGE('',*,*,#48208,.F.);
#64107=ORIENTED_EDGE('',*,*,#48229,.T.);
#64108=ORIENTED_EDGE('',*,*,#48210,.F.);
#64109=ORIENTED_EDGE('',*,*,#48230,.T.);
#64110=ORIENTED_EDGE('',*,*,#48231,.T.);
#64111=ORIENTED_EDGE('',*,*,#48232,.T.);
#64112=ORIENTED_EDGE('',*,*,#48233,.F.);
#64113=ORIENTED_EDGE('',*,*,#48234,.F.);
#64114=ORIENTED_EDGE('',*,*,#48235,.F.);
#64115=ORIENTED_EDGE('',*,*,#48236,.T.);
#64116=ORIENTED_EDGE('',*,*,#48234,.T.);
#64117=ORIENTED_EDGE('',*,*,#48237,.T.);
#64118=ORIENTED_EDGE('',*,*,#48238,.T.);
#64119=ORIENTED_EDGE('',*,*,#48239,.T.);
#64120=ORIENTED_EDGE('',*,*,#48240,.T.);
#64121=ORIENTED_EDGE('',*,*,#48241,.T.);
#64122=ORIENTED_EDGE('',*,*,#48242,.T.);
#64123=ORIENTED_EDGE('',*,*,#48243,.T.);
#64124=ORIENTED_EDGE('',*,*,#48244,.T.);
#64125=ORIENTED_EDGE('',*,*,#48245,.T.);
#64126=ORIENTED_EDGE('',*,*,#48246,.F.);
#64127=ORIENTED_EDGE('',*,*,#48247,.F.);
#64128=ORIENTED_EDGE('',*,*,#48248,.F.);
#64129=ORIENTED_EDGE('',*,*,#48249,.T.);
#64130=ORIENTED_EDGE('',*,*,#48247,.T.);
#64131=ORIENTED_EDGE('',*,*,#48250,.T.);
#64132=ORIENTED_EDGE('',*,*,#48251,.T.);
#64133=ORIENTED_EDGE('',*,*,#48252,.T.);
#64134=ORIENTED_EDGE('',*,*,#46416,.F.);
#64135=ORIENTED_EDGE('',*,*,#48253,.T.);
#64136=ORIENTED_EDGE('',*,*,#48231,.F.);
#64137=ORIENTED_EDGE('',*,*,#48254,.T.);
#64138=ORIENTED_EDGE('',*,*,#48251,.F.);
#64139=ORIENTED_EDGE('',*,*,#48255,.T.);
#64140=ORIENTED_EDGE('',*,*,#45956,.F.);
#64141=ORIENTED_EDGE('',*,*,#48256,.T.);
#64142=ORIENTED_EDGE('',*,*,#48242,.F.);
#64143=ORIENTED_EDGE('',*,*,#48257,.T.);
#64144=ORIENTED_EDGE('',*,*,#48244,.F.);
#64145=ORIENTED_EDGE('',*,*,#48258,.T.);
#64146=ORIENTED_EDGE('',*,*,#48238,.F.);
#64147=ORIENTED_EDGE('',*,*,#48259,.T.);
#64148=ORIENTED_EDGE('',*,*,#48240,.F.);
#64149=ORIENTED_EDGE('',*,*,#48260,.T.);
#64150=ORIENTED_EDGE('',*,*,#48261,.T.);
#64151=ORIENTED_EDGE('',*,*,#48262,.T.);
#64152=ORIENTED_EDGE('',*,*,#48263,.F.);
#64153=ORIENTED_EDGE('',*,*,#48264,.F.);
#64154=ORIENTED_EDGE('',*,*,#48265,.F.);
#64155=ORIENTED_EDGE('',*,*,#48266,.T.);
#64156=ORIENTED_EDGE('',*,*,#48264,.T.);
#64157=ORIENTED_EDGE('',*,*,#48267,.T.);
#64158=ORIENTED_EDGE('',*,*,#48268,.T.);
#64159=ORIENTED_EDGE('',*,*,#48269,.T.);
#64160=ORIENTED_EDGE('',*,*,#48270,.T.);
#64161=ORIENTED_EDGE('',*,*,#48271,.T.);
#64162=ORIENTED_EDGE('',*,*,#48272,.T.);
#64163=ORIENTED_EDGE('',*,*,#48273,.T.);
#64164=ORIENTED_EDGE('',*,*,#48274,.T.);
#64165=ORIENTED_EDGE('',*,*,#48275,.T.);
#64166=ORIENTED_EDGE('',*,*,#48276,.F.);
#64167=ORIENTED_EDGE('',*,*,#48277,.F.);
#64168=ORIENTED_EDGE('',*,*,#48278,.F.);
#64169=ORIENTED_EDGE('',*,*,#48279,.T.);
#64170=ORIENTED_EDGE('',*,*,#48277,.T.);
#64171=ORIENTED_EDGE('',*,*,#48280,.T.);
#64172=ORIENTED_EDGE('',*,*,#48281,.T.);
#64173=ORIENTED_EDGE('',*,*,#48282,.T.);
#64174=ORIENTED_EDGE('',*,*,#46422,.F.);
#64175=ORIENTED_EDGE('',*,*,#48283,.T.);
#64176=ORIENTED_EDGE('',*,*,#48261,.F.);
#64177=ORIENTED_EDGE('',*,*,#48284,.T.);
#64178=ORIENTED_EDGE('',*,*,#48281,.F.);
#64179=ORIENTED_EDGE('',*,*,#48285,.T.);
#64180=ORIENTED_EDGE('',*,*,#45950,.F.);
#64181=ORIENTED_EDGE('',*,*,#48286,.T.);
#64182=ORIENTED_EDGE('',*,*,#48272,.F.);
#64183=ORIENTED_EDGE('',*,*,#48287,.T.);
#64184=ORIENTED_EDGE('',*,*,#48274,.F.);
#64185=ORIENTED_EDGE('',*,*,#48288,.T.);
#64186=ORIENTED_EDGE('',*,*,#48268,.F.);
#64187=ORIENTED_EDGE('',*,*,#48289,.T.);
#64188=ORIENTED_EDGE('',*,*,#48270,.F.);
#64189=ORIENTED_EDGE('',*,*,#48290,.T.);
#64190=ORIENTED_EDGE('',*,*,#48291,.T.);
#64191=ORIENTED_EDGE('',*,*,#48292,.T.);
#64192=ORIENTED_EDGE('',*,*,#48293,.F.);
#64193=ORIENTED_EDGE('',*,*,#48294,.F.);
#64194=ORIENTED_EDGE('',*,*,#48295,.F.);
#64195=ORIENTED_EDGE('',*,*,#48296,.T.);
#64196=ORIENTED_EDGE('',*,*,#48294,.T.);
#64197=ORIENTED_EDGE('',*,*,#48297,.T.);
#64198=ORIENTED_EDGE('',*,*,#48298,.T.);
#64199=ORIENTED_EDGE('',*,*,#48299,.T.);
#64200=ORIENTED_EDGE('',*,*,#48300,.T.);
#64201=ORIENTED_EDGE('',*,*,#48301,.T.);
#64202=ORIENTED_EDGE('',*,*,#48302,.T.);
#64203=ORIENTED_EDGE('',*,*,#48303,.T.);
#64204=ORIENTED_EDGE('',*,*,#48304,.T.);
#64205=ORIENTED_EDGE('',*,*,#48305,.T.);
#64206=ORIENTED_EDGE('',*,*,#48306,.F.);
#64207=ORIENTED_EDGE('',*,*,#48307,.F.);
#64208=ORIENTED_EDGE('',*,*,#48308,.F.);
#64209=ORIENTED_EDGE('',*,*,#48309,.T.);
#64210=ORIENTED_EDGE('',*,*,#48307,.T.);
#64211=ORIENTED_EDGE('',*,*,#48310,.T.);
#64212=ORIENTED_EDGE('',*,*,#48311,.T.);
#64213=ORIENTED_EDGE('',*,*,#48312,.T.);
#64214=ORIENTED_EDGE('',*,*,#46428,.F.);
#64215=ORIENTED_EDGE('',*,*,#48313,.T.);
#64216=ORIENTED_EDGE('',*,*,#48291,.F.);
#64217=ORIENTED_EDGE('',*,*,#48314,.T.);
#64218=ORIENTED_EDGE('',*,*,#48311,.F.);
#64219=ORIENTED_EDGE('',*,*,#48315,.T.);
#64220=ORIENTED_EDGE('',*,*,#45944,.F.);
#64221=ORIENTED_EDGE('',*,*,#48316,.T.);
#64222=ORIENTED_EDGE('',*,*,#48302,.F.);
#64223=ORIENTED_EDGE('',*,*,#48317,.T.);
#64224=ORIENTED_EDGE('',*,*,#48304,.F.);
#64225=ORIENTED_EDGE('',*,*,#48318,.T.);
#64226=ORIENTED_EDGE('',*,*,#48298,.F.);
#64227=ORIENTED_EDGE('',*,*,#48319,.T.);
#64228=ORIENTED_EDGE('',*,*,#48300,.F.);
#64229=ORIENTED_EDGE('',*,*,#48320,.T.);
#64230=ORIENTED_EDGE('',*,*,#48321,.T.);
#64231=ORIENTED_EDGE('',*,*,#48322,.T.);
#64232=ORIENTED_EDGE('',*,*,#48323,.F.);
#64233=ORIENTED_EDGE('',*,*,#48324,.F.);
#64234=ORIENTED_EDGE('',*,*,#48325,.F.);
#64235=ORIENTED_EDGE('',*,*,#48326,.T.);
#64236=ORIENTED_EDGE('',*,*,#48324,.T.);
#64237=ORIENTED_EDGE('',*,*,#48327,.T.);
#64238=ORIENTED_EDGE('',*,*,#48328,.T.);
#64239=ORIENTED_EDGE('',*,*,#48329,.T.);
#64240=ORIENTED_EDGE('',*,*,#48330,.T.);
#64241=ORIENTED_EDGE('',*,*,#48331,.T.);
#64242=ORIENTED_EDGE('',*,*,#48332,.T.);
#64243=ORIENTED_EDGE('',*,*,#48333,.T.);
#64244=ORIENTED_EDGE('',*,*,#48334,.T.);
#64245=ORIENTED_EDGE('',*,*,#48335,.T.);
#64246=ORIENTED_EDGE('',*,*,#48336,.F.);
#64247=ORIENTED_EDGE('',*,*,#48337,.F.);
#64248=ORIENTED_EDGE('',*,*,#48338,.F.);
#64249=ORIENTED_EDGE('',*,*,#48339,.T.);
#64250=ORIENTED_EDGE('',*,*,#48337,.T.);
#64251=ORIENTED_EDGE('',*,*,#48340,.T.);
#64252=ORIENTED_EDGE('',*,*,#48341,.T.);
#64253=ORIENTED_EDGE('',*,*,#48342,.T.);
#64254=ORIENTED_EDGE('',*,*,#46434,.F.);
#64255=ORIENTED_EDGE('',*,*,#48343,.T.);
#64256=ORIENTED_EDGE('',*,*,#48321,.F.);
#64257=ORIENTED_EDGE('',*,*,#48344,.T.);
#64258=ORIENTED_EDGE('',*,*,#48341,.F.);
#64259=ORIENTED_EDGE('',*,*,#48345,.T.);
#64260=ORIENTED_EDGE('',*,*,#45938,.F.);
#64261=ORIENTED_EDGE('',*,*,#48346,.T.);
#64262=ORIENTED_EDGE('',*,*,#48332,.F.);
#64263=ORIENTED_EDGE('',*,*,#48347,.T.);
#64264=ORIENTED_EDGE('',*,*,#48334,.F.);
#64265=ORIENTED_EDGE('',*,*,#48348,.T.);
#64266=ORIENTED_EDGE('',*,*,#48328,.F.);
#64267=ORIENTED_EDGE('',*,*,#48349,.T.);
#64268=ORIENTED_EDGE('',*,*,#48330,.F.);
#64269=ORIENTED_EDGE('',*,*,#48350,.T.);
#64270=ORIENTED_EDGE('',*,*,#48351,.T.);
#64271=ORIENTED_EDGE('',*,*,#48352,.T.);
#64272=ORIENTED_EDGE('',*,*,#48353,.F.);
#64273=ORIENTED_EDGE('',*,*,#48354,.F.);
#64274=ORIENTED_EDGE('',*,*,#48355,.F.);
#64275=ORIENTED_EDGE('',*,*,#48356,.T.);
#64276=ORIENTED_EDGE('',*,*,#48354,.T.);
#64277=ORIENTED_EDGE('',*,*,#48357,.T.);
#64278=ORIENTED_EDGE('',*,*,#48358,.T.);
#64279=ORIENTED_EDGE('',*,*,#48359,.T.);
#64280=ORIENTED_EDGE('',*,*,#48360,.T.);
#64281=ORIENTED_EDGE('',*,*,#48361,.T.);
#64282=ORIENTED_EDGE('',*,*,#48362,.T.);
#64283=ORIENTED_EDGE('',*,*,#48363,.T.);
#64284=ORIENTED_EDGE('',*,*,#48364,.T.);
#64285=ORIENTED_EDGE('',*,*,#48365,.T.);
#64286=ORIENTED_EDGE('',*,*,#48366,.F.);
#64287=ORIENTED_EDGE('',*,*,#48367,.F.);
#64288=ORIENTED_EDGE('',*,*,#48368,.F.);
#64289=ORIENTED_EDGE('',*,*,#48369,.T.);
#64290=ORIENTED_EDGE('',*,*,#48367,.T.);
#64291=ORIENTED_EDGE('',*,*,#48370,.T.);
#64292=ORIENTED_EDGE('',*,*,#48371,.T.);
#64293=ORIENTED_EDGE('',*,*,#48372,.T.);
#64294=ORIENTED_EDGE('',*,*,#46440,.F.);
#64295=ORIENTED_EDGE('',*,*,#48373,.T.);
#64296=ORIENTED_EDGE('',*,*,#48351,.F.);
#64297=ORIENTED_EDGE('',*,*,#48374,.T.);
#64298=ORIENTED_EDGE('',*,*,#48371,.F.);
#64299=ORIENTED_EDGE('',*,*,#48375,.T.);
#64300=ORIENTED_EDGE('',*,*,#45932,.F.);
#64301=ORIENTED_EDGE('',*,*,#48376,.T.);
#64302=ORIENTED_EDGE('',*,*,#48362,.F.);
#64303=ORIENTED_EDGE('',*,*,#48377,.T.);
#64304=ORIENTED_EDGE('',*,*,#48364,.F.);
#64305=ORIENTED_EDGE('',*,*,#48378,.T.);
#64306=ORIENTED_EDGE('',*,*,#48358,.F.);
#64307=ORIENTED_EDGE('',*,*,#48379,.T.);
#64308=ORIENTED_EDGE('',*,*,#48360,.F.);
#64309=ORIENTED_EDGE('',*,*,#48380,.T.);
#64310=ORIENTED_EDGE('',*,*,#48381,.T.);
#64311=ORIENTED_EDGE('',*,*,#48382,.T.);
#64312=ORIENTED_EDGE('',*,*,#48383,.F.);
#64313=ORIENTED_EDGE('',*,*,#48384,.F.);
#64314=ORIENTED_EDGE('',*,*,#48385,.F.);
#64315=ORIENTED_EDGE('',*,*,#48386,.T.);
#64316=ORIENTED_EDGE('',*,*,#48384,.T.);
#64317=ORIENTED_EDGE('',*,*,#48387,.T.);
#64318=ORIENTED_EDGE('',*,*,#48388,.T.);
#64319=ORIENTED_EDGE('',*,*,#48389,.T.);
#64320=ORIENTED_EDGE('',*,*,#48390,.T.);
#64321=ORIENTED_EDGE('',*,*,#48391,.T.);
#64322=ORIENTED_EDGE('',*,*,#48392,.T.);
#64323=ORIENTED_EDGE('',*,*,#48393,.T.);
#64324=ORIENTED_EDGE('',*,*,#48394,.T.);
#64325=ORIENTED_EDGE('',*,*,#48395,.T.);
#64326=ORIENTED_EDGE('',*,*,#48396,.F.);
#64327=ORIENTED_EDGE('',*,*,#48397,.F.);
#64328=ORIENTED_EDGE('',*,*,#48398,.F.);
#64329=ORIENTED_EDGE('',*,*,#48399,.T.);
#64330=ORIENTED_EDGE('',*,*,#48397,.T.);
#64331=ORIENTED_EDGE('',*,*,#48400,.T.);
#64332=ORIENTED_EDGE('',*,*,#48401,.T.);
#64333=ORIENTED_EDGE('',*,*,#48402,.T.);
#64334=ORIENTED_EDGE('',*,*,#46446,.F.);
#64335=ORIENTED_EDGE('',*,*,#48403,.T.);
#64336=ORIENTED_EDGE('',*,*,#48381,.F.);
#64337=ORIENTED_EDGE('',*,*,#48404,.T.);
#64338=ORIENTED_EDGE('',*,*,#48401,.F.);
#64339=ORIENTED_EDGE('',*,*,#48405,.T.);
#64340=ORIENTED_EDGE('',*,*,#45926,.F.);
#64341=ORIENTED_EDGE('',*,*,#48406,.T.);
#64342=ORIENTED_EDGE('',*,*,#48392,.F.);
#64343=ORIENTED_EDGE('',*,*,#48407,.T.);
#64344=ORIENTED_EDGE('',*,*,#48394,.F.);
#64345=ORIENTED_EDGE('',*,*,#48408,.T.);
#64346=ORIENTED_EDGE('',*,*,#48388,.F.);
#64347=ORIENTED_EDGE('',*,*,#48409,.T.);
#64348=ORIENTED_EDGE('',*,*,#48390,.F.);
#64349=ORIENTED_EDGE('',*,*,#48410,.T.);
#64350=ORIENTED_EDGE('',*,*,#45905,.T.);
#64351=ORIENTED_EDGE('',*,*,#45899,.T.);
#64352=ORIENTED_EDGE('',*,*,#48411,.T.);
#64353=ORIENTED_EDGE('',*,*,#48412,.T.);
#64354=ORIENTED_EDGE('',*,*,#48413,.F.);
#64355=ORIENTED_EDGE('',*,*,#48414,.F.);
#64356=ORIENTED_EDGE('',*,*,#48415,.F.);
#64357=ORIENTED_EDGE('',*,*,#48416,.T.);
#64358=ORIENTED_EDGE('',*,*,#48414,.T.);
#64359=ORIENTED_EDGE('',*,*,#48417,.T.);
#64360=ORIENTED_EDGE('',*,*,#48418,.T.);
#64361=ORIENTED_EDGE('',*,*,#48419,.T.);
#64362=ORIENTED_EDGE('',*,*,#48420,.T.);
#64363=ORIENTED_EDGE('',*,*,#48421,.T.);
#64364=ORIENTED_EDGE('',*,*,#48422,.T.);
#64365=ORIENTED_EDGE('',*,*,#48423,.T.);
#64366=ORIENTED_EDGE('',*,*,#48424,.T.);
#64367=ORIENTED_EDGE('',*,*,#48425,.T.);
#64368=ORIENTED_EDGE('',*,*,#48426,.F.);
#64369=ORIENTED_EDGE('',*,*,#48427,.F.);
#64370=ORIENTED_EDGE('',*,*,#48428,.F.);
#64371=ORIENTED_EDGE('',*,*,#48429,.T.);
#64372=ORIENTED_EDGE('',*,*,#48427,.T.);
#64373=ORIENTED_EDGE('',*,*,#48430,.T.);
#64374=ORIENTED_EDGE('',*,*,#48431,.T.);
#64375=ORIENTED_EDGE('',*,*,#48432,.T.);
#64376=ORIENTED_EDGE('',*,*,#45912,.T.);
#64377=ORIENTED_EDGE('',*,*,#45906,.T.);
#64378=ORIENTED_EDGE('',*,*,#45913,.T.);
#64379=ORIENTED_EDGE('',*,*,#46640,.F.);
#64380=ORIENTED_EDGE('',*,*,#46452,.F.);
#64381=ORIENTED_EDGE('',*,*,#48433,.T.);
#64382=ORIENTED_EDGE('',*,*,#48411,.F.);
#64383=ORIENTED_EDGE('',*,*,#48434,.T.);
#64384=ORIENTED_EDGE('',*,*,#48431,.F.);
#64385=ORIENTED_EDGE('',*,*,#48435,.T.);
#64386=ORIENTED_EDGE('',*,*,#45920,.F.);
#64387=ORIENTED_EDGE('',*,*,#48436,.T.);
#64388=ORIENTED_EDGE('',*,*,#48422,.F.);
#64389=ORIENTED_EDGE('',*,*,#48437,.T.);
#64390=ORIENTED_EDGE('',*,*,#48424,.F.);
#64391=ORIENTED_EDGE('',*,*,#48438,.T.);
#64392=ORIENTED_EDGE('',*,*,#48418,.F.);
#64393=ORIENTED_EDGE('',*,*,#48439,.T.);
#64394=ORIENTED_EDGE('',*,*,#48420,.F.);
#64395=ORIENTED_EDGE('',*,*,#48440,.T.);
#64396=ORIENTED_EDGE('',*,*,#48441,.T.);
#64397=ORIENTED_EDGE('',*,*,#48442,.T.);
#64398=ORIENTED_EDGE('',*,*,#48443,.T.);
#64399=ORIENTED_EDGE('',*,*,#48444,.T.);
#64400=ORIENTED_EDGE('',*,*,#48445,.T.);
#64401=ORIENTED_EDGE('',*,*,#48446,.T.);
#64402=ORIENTED_EDGE('',*,*,#48447,.T.);
#64403=ORIENTED_EDGE('',*,*,#48448,.T.);
#64404=ORIENTED_EDGE('',*,*,#48449,.T.);
#64405=ORIENTED_EDGE('',*,*,#48450,.T.);
#64406=ORIENTED_EDGE('',*,*,#48451,.T.);
#64407=ORIENTED_EDGE('',*,*,#48452,.T.);
#64408=ORIENTED_EDGE('',*,*,#48453,.T.);
#64409=ORIENTED_EDGE('',*,*,#48454,.T.);
#64410=ORIENTED_EDGE('',*,*,#48455,.T.);
#64411=ORIENTED_EDGE('',*,*,#48456,.T.);
#64412=ORIENTED_EDGE('',*,*,#48457,.T.);
#64413=ORIENTED_EDGE('',*,*,#48458,.T.);
#64414=ORIENTED_EDGE('',*,*,#48459,.T.);
#64415=ORIENTED_EDGE('',*,*,#48460,.T.);
#64416=ORIENTED_EDGE('',*,*,#48461,.T.);
#64417=ORIENTED_EDGE('',*,*,#48462,.T.);
#64418=ORIENTED_EDGE('',*,*,#48463,.T.);
#64419=ORIENTED_EDGE('',*,*,#48464,.T.);
#64420=ORIENTED_EDGE('',*,*,#48465,.T.);
#64421=ORIENTED_EDGE('',*,*,#48466,.T.);
#64422=ORIENTED_EDGE('',*,*,#48467,.T.);
#64423=ORIENTED_EDGE('',*,*,#48468,.T.);
#64424=ORIENTED_EDGE('',*,*,#48459,.F.);
#64425=ORIENTED_EDGE('',*,*,#48469,.T.);
#64426=ORIENTED_EDGE('',*,*,#48441,.F.);
#64427=ORIENTED_EDGE('',*,*,#48470,.T.);
#64428=ORIENTED_EDGE('',*,*,#48443,.F.);
#64429=ORIENTED_EDGE('',*,*,#48471,.T.);
#64430=ORIENTED_EDGE('',*,*,#48447,.F.);
#64431=ORIENTED_EDGE('',*,*,#48472,.T.);
#64432=ORIENTED_EDGE('',*,*,#48473,.F.);
#64433=ORIENTED_EDGE('',*,*,#48467,.F.);
#64434=ORIENTED_EDGE('',*,*,#48474,.F.);
#64435=ORIENTED_EDGE('',*,*,#48429,.F.);
#64436=ORIENTED_EDGE('',*,*,#48474,.T.);
#64437=ORIENTED_EDGE('',*,*,#48466,.F.);
#64438=ORIENTED_EDGE('',*,*,#48475,.F.);
#64439=ORIENTED_EDGE('',*,*,#48438,.F.);
#64440=ORIENTED_EDGE('',*,*,#48428,.T.);
#64441=ORIENTED_EDGE('',*,*,#48432,.F.);
#64442=ORIENTED_EDGE('',*,*,#48476,.F.);
#64443=ORIENTED_EDGE('',*,*,#48468,.F.);
#64444=ORIENTED_EDGE('',*,*,#48473,.T.);
#64445=ORIENTED_EDGE('',*,*,#48475,.T.);
#64446=ORIENTED_EDGE('',*,*,#48465,.F.);
#64447=ORIENTED_EDGE('',*,*,#48477,.F.);
#64448=ORIENTED_EDGE('',*,*,#48423,.F.);
#64449=ORIENTED_EDGE('',*,*,#48476,.T.);
#64450=ORIENTED_EDGE('',*,*,#48436,.F.);
#64451=ORIENTED_EDGE('',*,*,#48478,.F.);
#64452=ORIENTED_EDGE('',*,*,#48457,.F.);
#64453=ORIENTED_EDGE('',*,*,#48477,.T.);
#64454=ORIENTED_EDGE('',*,*,#48464,.F.);
#64455=ORIENTED_EDGE('',*,*,#48479,.F.);
#64456=ORIENTED_EDGE('',*,*,#48440,.F.);
#64457=ORIENTED_EDGE('',*,*,#48478,.T.);
#64458=ORIENTED_EDGE('',*,*,#45919,.F.);
#64459=ORIENTED_EDGE('',*,*,#48480,.F.);
#64460=ORIENTED_EDGE('',*,*,#48458,.F.);
#64461=ORIENTED_EDGE('',*,*,#48479,.T.);
#64462=ORIENTED_EDGE('',*,*,#48463,.F.);
#64463=ORIENTED_EDGE('',*,*,#48481,.F.);
#64464=ORIENTED_EDGE('',*,*,#48415,.T.);
#64465=ORIENTED_EDGE('',*,*,#48419,.F.);
#64466=ORIENTED_EDGE('',*,*,#48480,.T.);
#64467=ORIENTED_EDGE('',*,*,#45918,.F.);
#64468=ORIENTED_EDGE('',*,*,#48482,.F.);
#64469=ORIENTED_EDGE('',*,*,#48469,.F.);
#64470=ORIENTED_EDGE('',*,*,#48481,.T.);
#64471=ORIENTED_EDGE('',*,*,#48462,.F.);
#64472=ORIENTED_EDGE('',*,*,#48483,.F.);
#64473=ORIENTED_EDGE('',*,*,#48416,.F.);
#64474=ORIENTED_EDGE('',*,*,#48482,.T.);
#64475=ORIENTED_EDGE('',*,*,#45917,.F.);
#64476=ORIENTED_EDGE('',*,*,#48484,.F.);
#64477=ORIENTED_EDGE('',*,*,#48442,.F.);
#64478=ORIENTED_EDGE('',*,*,#48483,.T.);
#64479=ORIENTED_EDGE('',*,*,#48461,.F.);
#64480=ORIENTED_EDGE('',*,*,#48485,.F.);
#64481=ORIENTED_EDGE('',*,*,#48434,.F.);
#64482=ORIENTED_EDGE('',*,*,#48484,.T.);
#64483=ORIENTED_EDGE('',*,*,#46275,.F.);
#64484=ORIENTED_EDGE('',*,*,#48486,.F.);
#64485=ORIENTED_EDGE('',*,*,#48471,.F.);
#64486=ORIENTED_EDGE('',*,*,#48485,.T.);
#64487=ORIENTED_EDGE('',*,*,#48460,.F.);
#64488=ORIENTED_EDGE('',*,*,#48487,.F.);
#64489=ORIENTED_EDGE('',*,*,#46453,.F.);
#64490=ORIENTED_EDGE('',*,*,#48486,.T.);
#64491=ORIENTED_EDGE('',*,*,#46274,.F.);
#64492=ORIENTED_EDGE('',*,*,#48488,.F.);
#64493=ORIENTED_EDGE('',*,*,#48448,.F.);
#64494=ORIENTED_EDGE('',*,*,#48487,.T.);
#64495=ORIENTED_EDGE('',*,*,#48470,.F.);
#64496=ORIENTED_EDGE('',*,*,#48489,.F.);
#64497=ORIENTED_EDGE('',*,*,#46454,.F.);
#64498=ORIENTED_EDGE('',*,*,#48488,.T.);
#64499=ORIENTED_EDGE('',*,*,#46666,.F.);
#64500=ORIENTED_EDGE('',*,*,#48490,.F.);
#64501=ORIENTED_EDGE('',*,*,#48449,.F.);
#64502=ORIENTED_EDGE('',*,*,#48489,.T.);
#64503=ORIENTED_EDGE('',*,*,#48444,.F.);
#64504=ORIENTED_EDGE('',*,*,#48491,.F.);
#64505=ORIENTED_EDGE('',*,*,#46457,.F.);
#64506=ORIENTED_EDGE('',*,*,#46455,.F.);
#64507=ORIENTED_EDGE('',*,*,#46662,.F.);
#64508=ORIENTED_EDGE('',*,*,#46658,.T.);
#64509=ORIENTED_EDGE('',*,*,#48492,.F.);
#64510=ORIENTED_EDGE('',*,*,#48450,.F.);
#64511=ORIENTED_EDGE('',*,*,#48490,.T.);
#64512=ORIENTED_EDGE('',*,*,#48491,.T.);
#64513=ORIENTED_EDGE('',*,*,#48472,.F.);
#64514=ORIENTED_EDGE('',*,*,#48493,.F.);
#64515=ORIENTED_EDGE('',*,*,#46458,.F.);
#64516=ORIENTED_EDGE('',*,*,#48492,.T.);
#64517=ORIENTED_EDGE('',*,*,#46657,.F.);
#64518=ORIENTED_EDGE('',*,*,#48494,.F.);
#64519=ORIENTED_EDGE('',*,*,#48451,.F.);
#64520=ORIENTED_EDGE('',*,*,#48493,.T.);
#64521=ORIENTED_EDGE('',*,*,#48446,.F.);
#64522=ORIENTED_EDGE('',*,*,#48495,.F.);
#64523=ORIENTED_EDGE('',*,*,#46459,.F.);
#64524=ORIENTED_EDGE('',*,*,#48494,.T.);
#64525=ORIENTED_EDGE('',*,*,#46668,.F.);
#64526=ORIENTED_EDGE('',*,*,#48496,.F.);
#64527=ORIENTED_EDGE('',*,*,#48452,.F.);
#64528=ORIENTED_EDGE('',*,*,#48495,.T.);
#64529=ORIENTED_EDGE('',*,*,#48445,.F.);
#64530=ORIENTED_EDGE('',*,*,#48497,.F.);
#64531=ORIENTED_EDGE('',*,*,#46664,.F.);
#64532=ORIENTED_EDGE('',*,*,#48496,.T.);
#64533=ORIENTED_EDGE('',*,*,#46653,.F.);
#64534=ORIENTED_EDGE('',*,*,#48498,.F.);
#64535=ORIENTED_EDGE('',*,*,#48453,.F.);
#64536=ORIENTED_EDGE('',*,*,#48497,.T.);
#64537=ORIENTED_EDGE('',*,*,#48456,.F.);
#64538=ORIENTED_EDGE('',*,*,#48499,.F.);
#64539=ORIENTED_EDGE('',*,*,#46644,.F.);
#64540=ORIENTED_EDGE('',*,*,#48498,.T.);
#64541=ORIENTED_EDGE('',*,*,#46670,.F.);
#64542=ORIENTED_EDGE('',*,*,#48500,.F.);
#64543=ORIENTED_EDGE('',*,*,#48454,.F.);
#64544=ORIENTED_EDGE('',*,*,#48499,.T.);
#64545=ORIENTED_EDGE('',*,*,#48455,.F.);
#64546=ORIENTED_EDGE('',*,*,#48500,.T.);
#64547=ORIENTED_EDGE('',*,*,#46649,.F.);
#64548=ORIENTED_EDGE('',*,*,#46645,.T.);
#64549=ORIENTED_EDGE('',*,*,#48501,.T.);
#64550=ORIENTED_EDGE('',*,*,#48502,.T.);
#64551=ORIENTED_EDGE('',*,*,#48503,.T.);
#64552=ORIENTED_EDGE('',*,*,#48504,.T.);
#64553=ORIENTED_EDGE('',*,*,#48505,.T.);
#64554=ORIENTED_EDGE('',*,*,#48506,.T.);
#64555=ORIENTED_EDGE('',*,*,#48507,.T.);
#64556=ORIENTED_EDGE('',*,*,#48508,.T.);
#64557=ORIENTED_EDGE('',*,*,#48509,.T.);
#64558=ORIENTED_EDGE('',*,*,#48510,.T.);
#64559=ORIENTED_EDGE('',*,*,#48511,.T.);
#64560=ORIENTED_EDGE('',*,*,#48512,.T.);
#64561=ORIENTED_EDGE('',*,*,#48513,.T.);
#64562=ORIENTED_EDGE('',*,*,#48514,.T.);
#64563=ORIENTED_EDGE('',*,*,#48515,.T.);
#64564=ORIENTED_EDGE('',*,*,#48516,.T.);
#64565=ORIENTED_EDGE('',*,*,#48517,.T.);
#64566=ORIENTED_EDGE('',*,*,#48518,.T.);
#64567=ORIENTED_EDGE('',*,*,#48519,.T.);
#64568=ORIENTED_EDGE('',*,*,#48520,.T.);
#64569=ORIENTED_EDGE('',*,*,#48521,.T.);
#64570=ORIENTED_EDGE('',*,*,#48522,.T.);
#64571=ORIENTED_EDGE('',*,*,#48523,.T.);
#64572=ORIENTED_EDGE('',*,*,#48524,.T.);
#64573=ORIENTED_EDGE('',*,*,#48525,.T.);
#64574=ORIENTED_EDGE('',*,*,#48526,.T.);
#64575=ORIENTED_EDGE('',*,*,#48527,.T.);
#64576=ORIENTED_EDGE('',*,*,#48528,.T.);
#64577=ORIENTED_EDGE('',*,*,#48529,.T.);
#64578=ORIENTED_EDGE('',*,*,#48530,.T.);
#64579=ORIENTED_EDGE('',*,*,#48531,.T.);
#64580=ORIENTED_EDGE('',*,*,#48532,.T.);
#64581=ORIENTED_EDGE('',*,*,#48533,.T.);
#64582=ORIENTED_EDGE('',*,*,#48534,.T.);
#64583=ORIENTED_EDGE('',*,*,#48535,.T.);
#64584=ORIENTED_EDGE('',*,*,#48536,.T.);
#64585=ORIENTED_EDGE('',*,*,#48537,.T.);
#64586=ORIENTED_EDGE('',*,*,#48538,.T.);
#64587=ORIENTED_EDGE('',*,*,#48539,.T.);
#64588=ORIENTED_EDGE('',*,*,#48540,.T.);
#64589=ORIENTED_EDGE('',*,*,#48541,.T.);
#64590=ORIENTED_EDGE('',*,*,#48542,.T.);
#64591=ORIENTED_EDGE('',*,*,#48543,.T.);
#64592=ORIENTED_EDGE('',*,*,#48544,.T.);
#64593=ORIENTED_EDGE('',*,*,#48545,.T.);
#64594=ORIENTED_EDGE('',*,*,#48546,.T.);
#64595=ORIENTED_EDGE('',*,*,#48547,.T.);
#64596=ORIENTED_EDGE('',*,*,#48548,.T.);
#64597=ORIENTED_EDGE('',*,*,#48549,.T.);
#64598=ORIENTED_EDGE('',*,*,#48550,.T.);
#64599=ORIENTED_EDGE('',*,*,#48551,.T.);
#64600=ORIENTED_EDGE('',*,*,#48552,.T.);
#64601=ORIENTED_EDGE('',*,*,#48553,.T.);
#64602=ORIENTED_EDGE('',*,*,#48554,.T.);
#64603=ORIENTED_EDGE('',*,*,#48555,.T.);
#64604=ORIENTED_EDGE('',*,*,#48556,.T.);
#64605=ORIENTED_EDGE('',*,*,#48557,.T.);
#64606=ORIENTED_EDGE('',*,*,#48558,.T.);
#64607=ORIENTED_EDGE('',*,*,#48559,.T.);
#64608=ORIENTED_EDGE('',*,*,#48560,.T.);
#64609=ORIENTED_EDGE('',*,*,#48561,.T.);
#64610=ORIENTED_EDGE('',*,*,#48562,.T.);
#64611=ORIENTED_EDGE('',*,*,#48563,.T.);
#64612=ORIENTED_EDGE('',*,*,#48564,.T.);
#64613=ORIENTED_EDGE('',*,*,#48565,.T.);
#64614=ORIENTED_EDGE('',*,*,#48566,.T.);
#64615=ORIENTED_EDGE('',*,*,#48567,.T.);
#64616=ORIENTED_EDGE('',*,*,#48568,.T.);
#64617=ORIENTED_EDGE('',*,*,#48569,.T.);
#64618=ORIENTED_EDGE('',*,*,#48570,.T.);
#64619=ORIENTED_EDGE('',*,*,#48571,.T.);
#64620=ORIENTED_EDGE('',*,*,#48572,.T.);
#64621=ORIENTED_EDGE('',*,*,#48573,.T.);
#64622=ORIENTED_EDGE('',*,*,#48574,.T.);
#64623=ORIENTED_EDGE('',*,*,#48575,.T.);
#64624=ORIENTED_EDGE('',*,*,#48576,.T.);
#64625=ORIENTED_EDGE('',*,*,#48577,.T.);
#64626=ORIENTED_EDGE('',*,*,#48578,.T.);
#64627=ORIENTED_EDGE('',*,*,#48579,.T.);
#64628=ORIENTED_EDGE('',*,*,#48580,.T.);
#64629=ORIENTED_EDGE('',*,*,#48581,.T.);
#64630=ORIENTED_EDGE('',*,*,#48582,.T.);
#64631=ORIENTED_EDGE('',*,*,#48583,.T.);
#64632=ORIENTED_EDGE('',*,*,#48584,.T.);
#64633=ORIENTED_EDGE('',*,*,#48585,.T.);
#64634=ORIENTED_EDGE('',*,*,#48586,.T.);
#64635=ORIENTED_EDGE('',*,*,#48587,.T.);
#64636=ORIENTED_EDGE('',*,*,#48588,.T.);
#64637=ORIENTED_EDGE('',*,*,#48589,.T.);
#64638=ORIENTED_EDGE('',*,*,#48590,.T.);
#64639=ORIENTED_EDGE('',*,*,#48591,.T.);
#64640=ORIENTED_EDGE('',*,*,#48592,.T.);
#64641=ORIENTED_EDGE('',*,*,#48593,.T.);
#64642=ORIENTED_EDGE('',*,*,#48594,.T.);
#64643=ORIENTED_EDGE('',*,*,#48595,.T.);
#64644=ORIENTED_EDGE('',*,*,#48596,.T.);
#64645=ORIENTED_EDGE('',*,*,#48597,.T.);
#64646=ORIENTED_EDGE('',*,*,#48598,.T.);
#64647=ORIENTED_EDGE('',*,*,#48599,.T.);
#64648=ORIENTED_EDGE('',*,*,#48600,.T.);
#64649=ORIENTED_EDGE('',*,*,#48601,.T.);
#64650=ORIENTED_EDGE('',*,*,#48602,.T.);
#64651=ORIENTED_EDGE('',*,*,#48603,.T.);
#64652=ORIENTED_EDGE('',*,*,#48604,.T.);
#64653=ORIENTED_EDGE('',*,*,#48605,.T.);
#64654=ORIENTED_EDGE('',*,*,#48606,.T.);
#64655=ORIENTED_EDGE('',*,*,#48607,.T.);
#64656=ORIENTED_EDGE('',*,*,#48608,.T.);
#64657=ORIENTED_EDGE('',*,*,#48609,.T.);
#64658=ORIENTED_EDGE('',*,*,#48610,.T.);
#64659=ORIENTED_EDGE('',*,*,#48611,.T.);
#64660=ORIENTED_EDGE('',*,*,#48612,.T.);
#64661=ORIENTED_EDGE('',*,*,#48613,.T.);
#64662=ORIENTED_EDGE('',*,*,#48614,.T.);
#64663=ORIENTED_EDGE('',*,*,#48615,.T.);
#64664=ORIENTED_EDGE('',*,*,#48616,.T.);
#64665=ORIENTED_EDGE('',*,*,#48617,.T.);
#64666=ORIENTED_EDGE('',*,*,#48618,.T.);
#64667=ORIENTED_EDGE('',*,*,#48619,.T.);
#64668=ORIENTED_EDGE('',*,*,#48620,.T.);
#64669=ORIENTED_EDGE('',*,*,#48621,.T.);
#64670=ORIENTED_EDGE('',*,*,#48622,.T.);
#64671=ORIENTED_EDGE('',*,*,#48623,.T.);
#64672=ORIENTED_EDGE('',*,*,#48624,.T.);
#64673=ORIENTED_EDGE('',*,*,#48625,.T.);
#64674=ORIENTED_EDGE('',*,*,#48626,.T.);
#64675=ORIENTED_EDGE('',*,*,#48627,.T.);
#64676=ORIENTED_EDGE('',*,*,#48628,.T.);
#64677=ORIENTED_EDGE('',*,*,#48629,.T.);
#64678=ORIENTED_EDGE('',*,*,#48630,.T.);
#64679=ORIENTED_EDGE('',*,*,#48631,.T.);
#64680=ORIENTED_EDGE('',*,*,#48632,.T.);
#64681=ORIENTED_EDGE('',*,*,#48633,.T.);
#64682=ORIENTED_EDGE('',*,*,#48634,.T.);
#64683=ORIENTED_EDGE('',*,*,#48635,.T.);
#64684=ORIENTED_EDGE('',*,*,#48636,.T.);
#64685=ORIENTED_EDGE('',*,*,#48637,.T.);
#64686=ORIENTED_EDGE('',*,*,#48638,.T.);
#64687=ORIENTED_EDGE('',*,*,#48639,.T.);
#64688=ORIENTED_EDGE('',*,*,#48640,.T.);
#64689=ORIENTED_EDGE('',*,*,#48641,.T.);
#64690=ORIENTED_EDGE('',*,*,#48642,.T.);
#64691=ORIENTED_EDGE('',*,*,#48643,.T.);
#64692=ORIENTED_EDGE('',*,*,#48644,.T.);
#64693=ORIENTED_EDGE('',*,*,#48645,.T.);
#64694=ORIENTED_EDGE('',*,*,#48646,.T.);
#64695=ORIENTED_EDGE('',*,*,#48647,.T.);
#64696=ORIENTED_EDGE('',*,*,#48648,.T.);
#64697=ORIENTED_EDGE('',*,*,#48649,.T.);
#64698=ORIENTED_EDGE('',*,*,#48650,.T.);
#64699=ORIENTED_EDGE('',*,*,#48651,.T.);
#64700=ORIENTED_EDGE('',*,*,#48652,.T.);
#64701=ORIENTED_EDGE('',*,*,#48653,.T.);
#64702=ORIENTED_EDGE('',*,*,#48654,.T.);
#64703=ORIENTED_EDGE('',*,*,#48655,.T.);
#64704=ORIENTED_EDGE('',*,*,#48656,.T.);
#64705=ORIENTED_EDGE('',*,*,#48657,.T.);
#64706=ORIENTED_EDGE('',*,*,#48658,.T.);
#64707=ORIENTED_EDGE('',*,*,#48659,.T.);
#64708=ORIENTED_EDGE('',*,*,#48660,.T.);
#64709=ORIENTED_EDGE('',*,*,#48661,.T.);
#64710=ORIENTED_EDGE('',*,*,#48662,.T.);
#64711=ORIENTED_EDGE('',*,*,#48663,.T.);
#64712=ORIENTED_EDGE('',*,*,#48664,.T.);
#64713=ORIENTED_EDGE('',*,*,#48665,.T.);
#64714=ORIENTED_EDGE('',*,*,#48666,.T.);
#64715=ORIENTED_EDGE('',*,*,#48667,.T.);
#64716=ORIENTED_EDGE('',*,*,#48668,.T.);
#64717=ORIENTED_EDGE('',*,*,#48669,.T.);
#64718=ORIENTED_EDGE('',*,*,#48670,.T.);
#64719=ORIENTED_EDGE('',*,*,#48671,.T.);
#64720=ORIENTED_EDGE('',*,*,#48672,.T.);
#64721=ORIENTED_EDGE('',*,*,#48673,.T.);
#64722=ORIENTED_EDGE('',*,*,#48674,.T.);
#64723=ORIENTED_EDGE('',*,*,#48675,.T.);
#64724=ORIENTED_EDGE('',*,*,#48676,.T.);
#64725=ORIENTED_EDGE('',*,*,#48677,.T.);
#64726=ORIENTED_EDGE('',*,*,#48678,.T.);
#64727=ORIENTED_EDGE('',*,*,#48679,.T.);
#64728=ORIENTED_EDGE('',*,*,#48680,.T.);
#64729=ORIENTED_EDGE('',*,*,#48681,.T.);
#64730=ORIENTED_EDGE('',*,*,#48682,.T.);
#64731=ORIENTED_EDGE('',*,*,#48683,.T.);
#64732=ORIENTED_EDGE('',*,*,#48684,.T.);
#64733=ORIENTED_EDGE('',*,*,#48685,.T.);
#64734=ORIENTED_EDGE('',*,*,#48686,.T.);
#64735=ORIENTED_EDGE('',*,*,#48687,.T.);
#64736=ORIENTED_EDGE('',*,*,#48688,.T.);
#64737=ORIENTED_EDGE('',*,*,#48689,.T.);
#64738=ORIENTED_EDGE('',*,*,#48690,.T.);
#64739=ORIENTED_EDGE('',*,*,#48691,.T.);
#64740=ORIENTED_EDGE('',*,*,#48692,.T.);
#64741=ORIENTED_EDGE('',*,*,#48693,.T.);
#64742=ORIENTED_EDGE('',*,*,#48694,.T.);
#64743=ORIENTED_EDGE('',*,*,#48695,.T.);
#64744=ORIENTED_EDGE('',*,*,#48696,.T.);
#64745=ORIENTED_EDGE('',*,*,#48697,.T.);
#64746=ORIENTED_EDGE('',*,*,#48698,.T.);
#64747=ORIENTED_EDGE('',*,*,#48699,.T.);
#64748=ORIENTED_EDGE('',*,*,#48700,.T.);
#64749=ORIENTED_EDGE('',*,*,#48701,.T.);
#64750=ORIENTED_EDGE('',*,*,#48702,.T.);
#64751=ORIENTED_EDGE('',*,*,#48703,.T.);
#64752=ORIENTED_EDGE('',*,*,#48704,.T.);
#64753=ORIENTED_EDGE('',*,*,#48705,.T.);
#64754=ORIENTED_EDGE('',*,*,#48706,.T.);
#64755=ORIENTED_EDGE('',*,*,#48707,.T.);
#64756=ORIENTED_EDGE('',*,*,#48708,.T.);
#64757=ORIENTED_EDGE('',*,*,#48709,.T.);
#64758=ORIENTED_EDGE('',*,*,#48710,.T.);
#64759=ORIENTED_EDGE('',*,*,#48711,.T.);
#64760=ORIENTED_EDGE('',*,*,#48712,.T.);
#64761=ORIENTED_EDGE('',*,*,#48713,.T.);
#64762=ORIENTED_EDGE('',*,*,#48714,.T.);
#64763=ORIENTED_EDGE('',*,*,#48715,.T.);
#64764=ORIENTED_EDGE('',*,*,#48716,.T.);
#64765=ORIENTED_EDGE('',*,*,#48717,.T.);
#64766=ORIENTED_EDGE('',*,*,#48718,.T.);
#64767=ORIENTED_EDGE('',*,*,#48719,.T.);
#64768=ORIENTED_EDGE('',*,*,#48720,.T.);
#64769=ORIENTED_EDGE('',*,*,#48721,.T.);
#64770=ORIENTED_EDGE('',*,*,#48722,.T.);
#64771=ORIENTED_EDGE('',*,*,#48723,.T.);
#64772=ORIENTED_EDGE('',*,*,#48724,.T.);
#64773=ORIENTED_EDGE('',*,*,#48725,.T.);
#64774=ORIENTED_EDGE('',*,*,#48726,.T.);
#64775=ORIENTED_EDGE('',*,*,#48727,.T.);
#64776=ORIENTED_EDGE('',*,*,#48728,.T.);
#64777=ORIENTED_EDGE('',*,*,#48729,.T.);
#64778=ORIENTED_EDGE('',*,*,#48730,.T.);
#64779=ORIENTED_EDGE('',*,*,#48731,.T.);
#64780=ORIENTED_EDGE('',*,*,#48732,.T.);
#64781=ORIENTED_EDGE('',*,*,#48733,.T.);
#64782=ORIENTED_EDGE('',*,*,#48734,.T.);
#64783=ORIENTED_EDGE('',*,*,#48735,.T.);
#64784=ORIENTED_EDGE('',*,*,#48736,.T.);
#64785=ORIENTED_EDGE('',*,*,#48737,.T.);
#64786=ORIENTED_EDGE('',*,*,#48738,.T.);
#64787=ORIENTED_EDGE('',*,*,#48739,.T.);
#64788=ORIENTED_EDGE('',*,*,#48740,.T.);
#64789=ORIENTED_EDGE('',*,*,#48741,.T.);
#64790=ORIENTED_EDGE('',*,*,#48742,.T.);
#64791=ORIENTED_EDGE('',*,*,#48743,.T.);
#64792=ORIENTED_EDGE('',*,*,#48744,.T.);
#64793=ORIENTED_EDGE('',*,*,#48745,.T.);
#64794=ORIENTED_EDGE('',*,*,#48746,.T.);
#64795=ORIENTED_EDGE('',*,*,#48747,.T.);
#64796=ORIENTED_EDGE('',*,*,#48748,.T.);
#64797=ORIENTED_EDGE('',*,*,#48749,.T.);
#64798=ORIENTED_EDGE('',*,*,#48750,.T.);
#64799=ORIENTED_EDGE('',*,*,#48751,.T.);
#64800=ORIENTED_EDGE('',*,*,#48752,.T.);
#64801=ORIENTED_EDGE('',*,*,#48753,.T.);
#64802=ORIENTED_EDGE('',*,*,#48754,.T.);
#64803=ORIENTED_EDGE('',*,*,#48755,.T.);
#64804=ORIENTED_EDGE('',*,*,#48756,.T.);
#64805=ORIENTED_EDGE('',*,*,#48757,.T.);
#64806=ORIENTED_EDGE('',*,*,#48758,.T.);
#64807=ORIENTED_EDGE('',*,*,#48759,.T.);
#64808=ORIENTED_EDGE('',*,*,#48760,.T.);
#64809=ORIENTED_EDGE('',*,*,#48761,.T.);
#64810=ORIENTED_EDGE('',*,*,#48762,.T.);
#64811=ORIENTED_EDGE('',*,*,#48763,.T.);
#64812=ORIENTED_EDGE('',*,*,#48764,.T.);
#64813=ORIENTED_EDGE('',*,*,#48765,.T.);
#64814=ORIENTED_EDGE('',*,*,#48766,.T.);
#64815=ORIENTED_EDGE('',*,*,#48767,.T.);
#64816=ORIENTED_EDGE('',*,*,#48768,.T.);
#64817=ORIENTED_EDGE('',*,*,#48769,.T.);
#64818=ORIENTED_EDGE('',*,*,#48770,.T.);
#64819=ORIENTED_EDGE('',*,*,#48771,.T.);
#64820=ORIENTED_EDGE('',*,*,#48772,.T.);
#64821=ORIENTED_EDGE('',*,*,#48773,.T.);
#64822=ORIENTED_EDGE('',*,*,#48774,.T.);
#64823=ORIENTED_EDGE('',*,*,#48775,.T.);
#64824=ORIENTED_EDGE('',*,*,#48776,.T.);
#64825=ORIENTED_EDGE('',*,*,#48777,.T.);
#64826=ORIENTED_EDGE('',*,*,#48778,.T.);
#64827=ORIENTED_EDGE('',*,*,#48779,.T.);
#64828=ORIENTED_EDGE('',*,*,#48780,.T.);
#64829=ORIENTED_EDGE('',*,*,#48781,.T.);
#64830=ORIENTED_EDGE('',*,*,#48782,.T.);
#64831=ORIENTED_EDGE('',*,*,#48783,.T.);
#64832=ORIENTED_EDGE('',*,*,#48784,.T.);
#64833=ORIENTED_EDGE('',*,*,#48785,.T.);
#64834=ORIENTED_EDGE('',*,*,#48786,.T.);
#64835=ORIENTED_EDGE('',*,*,#48787,.T.);
#64836=ORIENTED_EDGE('',*,*,#48788,.T.);
#64837=ORIENTED_EDGE('',*,*,#48789,.T.);
#64838=ORIENTED_EDGE('',*,*,#48790,.T.);
#64839=ORIENTED_EDGE('',*,*,#48791,.T.);
#64840=ORIENTED_EDGE('',*,*,#48792,.T.);
#64841=ORIENTED_EDGE('',*,*,#48793,.T.);
#64842=ORIENTED_EDGE('',*,*,#48794,.T.);
#64843=ORIENTED_EDGE('',*,*,#48795,.T.);
#64844=ORIENTED_EDGE('',*,*,#48796,.T.);
#64845=ORIENTED_EDGE('',*,*,#48797,.T.);
#64846=ORIENTED_EDGE('',*,*,#48798,.T.);
#64847=ORIENTED_EDGE('',*,*,#48799,.T.);
#64848=ORIENTED_EDGE('',*,*,#48800,.T.);
#64849=ORIENTED_EDGE('',*,*,#48801,.T.);
#64850=ORIENTED_EDGE('',*,*,#48802,.T.);
#64851=ORIENTED_EDGE('',*,*,#48803,.T.);
#64852=ORIENTED_EDGE('',*,*,#48804,.T.);
#64853=ORIENTED_EDGE('',*,*,#48805,.T.);
#64854=ORIENTED_EDGE('',*,*,#48806,.T.);
#64855=ORIENTED_EDGE('',*,*,#48807,.T.);
#64856=ORIENTED_EDGE('',*,*,#48808,.T.);
#64857=ORIENTED_EDGE('',*,*,#48809,.T.);
#64858=ORIENTED_EDGE('',*,*,#48810,.T.);
#64859=ORIENTED_EDGE('',*,*,#48811,.T.);
#64860=ORIENTED_EDGE('',*,*,#48812,.T.);
#64861=ORIENTED_EDGE('',*,*,#48813,.T.);
#64862=ORIENTED_EDGE('',*,*,#48814,.T.);
#64863=ORIENTED_EDGE('',*,*,#48815,.T.);
#64864=ORIENTED_EDGE('',*,*,#48816,.T.);
#64865=ORIENTED_EDGE('',*,*,#48817,.T.);
#64866=ORIENTED_EDGE('',*,*,#48818,.T.);
#64867=ORIENTED_EDGE('',*,*,#48819,.T.);
#64868=ORIENTED_EDGE('',*,*,#48820,.T.);
#64869=ORIENTED_EDGE('',*,*,#48821,.T.);
#64870=ORIENTED_EDGE('',*,*,#48822,.T.);
#64871=ORIENTED_EDGE('',*,*,#48823,.T.);
#64872=ORIENTED_EDGE('',*,*,#48824,.T.);
#64873=ORIENTED_EDGE('',*,*,#48825,.T.);
#64874=ORIENTED_EDGE('',*,*,#48826,.T.);
#64875=ORIENTED_EDGE('',*,*,#48827,.T.);
#64876=ORIENTED_EDGE('',*,*,#48828,.T.);
#64877=ORIENTED_EDGE('',*,*,#48829,.T.);
#64878=ORIENTED_EDGE('',*,*,#48830,.T.);
#64879=ORIENTED_EDGE('',*,*,#48831,.T.);
#64880=ORIENTED_EDGE('',*,*,#48832,.T.);
#64881=ORIENTED_EDGE('',*,*,#48833,.T.);
#64882=ORIENTED_EDGE('',*,*,#48834,.T.);
#64883=ORIENTED_EDGE('',*,*,#48835,.T.);
#64884=ORIENTED_EDGE('',*,*,#48836,.T.);
#64885=ORIENTED_EDGE('',*,*,#48837,.T.);
#64886=ORIENTED_EDGE('',*,*,#48838,.T.);
#64887=ORIENTED_EDGE('',*,*,#48839,.T.);
#64888=ORIENTED_EDGE('',*,*,#48840,.T.);
#64889=ORIENTED_EDGE('',*,*,#48841,.T.);
#64890=ORIENTED_EDGE('',*,*,#48842,.T.);
#64891=ORIENTED_EDGE('',*,*,#48843,.T.);
#64892=ORIENTED_EDGE('',*,*,#48844,.T.);
#64893=ORIENTED_EDGE('',*,*,#48845,.T.);
#64894=ORIENTED_EDGE('',*,*,#48846,.T.);
#64895=ORIENTED_EDGE('',*,*,#48847,.T.);
#64896=ORIENTED_EDGE('',*,*,#48848,.T.);
#64897=ORIENTED_EDGE('',*,*,#48849,.T.);
#64898=ORIENTED_EDGE('',*,*,#48850,.T.);
#64899=ORIENTED_EDGE('',*,*,#48851,.T.);
#64900=ORIENTED_EDGE('',*,*,#48852,.T.);
#64901=ORIENTED_EDGE('',*,*,#48853,.T.);
#64902=ORIENTED_EDGE('',*,*,#48854,.T.);
#64903=ORIENTED_EDGE('',*,*,#48855,.T.);
#64904=ORIENTED_EDGE('',*,*,#48856,.T.);
#64905=ORIENTED_EDGE('',*,*,#48857,.T.);
#64906=ORIENTED_EDGE('',*,*,#48858,.T.);
#64907=ORIENTED_EDGE('',*,*,#48859,.T.);
#64908=ORIENTED_EDGE('',*,*,#48860,.T.);
#64909=ORIENTED_EDGE('',*,*,#48861,.T.);
#64910=ORIENTED_EDGE('',*,*,#48862,.T.);
#64911=ORIENTED_EDGE('',*,*,#48863,.T.);
#64912=ORIENTED_EDGE('',*,*,#48864,.T.);
#64913=ORIENTED_EDGE('',*,*,#48865,.T.);
#64914=ORIENTED_EDGE('',*,*,#48866,.T.);
#64915=ORIENTED_EDGE('',*,*,#48867,.T.);
#64916=ORIENTED_EDGE('',*,*,#48868,.T.);
#64917=ORIENTED_EDGE('',*,*,#48869,.T.);
#64918=ORIENTED_EDGE('',*,*,#48870,.T.);
#64919=ORIENTED_EDGE('',*,*,#48871,.T.);
#64920=ORIENTED_EDGE('',*,*,#48872,.T.);
#64921=ORIENTED_EDGE('',*,*,#48873,.T.);
#64922=ORIENTED_EDGE('',*,*,#48874,.T.);
#64923=ORIENTED_EDGE('',*,*,#48875,.T.);
#64924=ORIENTED_EDGE('',*,*,#48876,.T.);
#64925=ORIENTED_EDGE('',*,*,#48877,.T.);
#64926=ORIENTED_EDGE('',*,*,#48878,.T.);
#64927=ORIENTED_EDGE('',*,*,#48879,.T.);
#64928=ORIENTED_EDGE('',*,*,#48880,.T.);
#64929=ORIENTED_EDGE('',*,*,#48881,.T.);
#64930=ORIENTED_EDGE('',*,*,#48882,.T.);
#64931=ORIENTED_EDGE('',*,*,#48883,.T.);
#64932=ORIENTED_EDGE('',*,*,#48884,.T.);
#64933=ORIENTED_EDGE('',*,*,#48885,.T.);
#64934=ORIENTED_EDGE('',*,*,#48886,.T.);
#64935=ORIENTED_EDGE('',*,*,#48887,.T.);
#64936=ORIENTED_EDGE('',*,*,#48888,.T.);
#64937=ORIENTED_EDGE('',*,*,#48889,.T.);
#64938=ORIENTED_EDGE('',*,*,#48890,.T.);
#64939=ORIENTED_EDGE('',*,*,#48891,.T.);
#64940=ORIENTED_EDGE('',*,*,#48892,.T.);
#64941=ORIENTED_EDGE('',*,*,#48893,.T.);
#64942=ORIENTED_EDGE('',*,*,#48894,.T.);
#64943=ORIENTED_EDGE('',*,*,#48895,.T.);
#64944=ORIENTED_EDGE('',*,*,#48896,.T.);
#64945=ORIENTED_EDGE('',*,*,#48897,.T.);
#64946=ORIENTED_EDGE('',*,*,#48898,.T.);
#64947=ORIENTED_EDGE('',*,*,#48899,.T.);
#64948=ORIENTED_EDGE('',*,*,#48900,.T.);
#64949=ORIENTED_EDGE('',*,*,#48901,.T.);
#64950=ORIENTED_EDGE('',*,*,#48902,.T.);
#64951=ORIENTED_EDGE('',*,*,#48903,.T.);
#64952=ORIENTED_EDGE('',*,*,#48904,.T.);
#64953=ORIENTED_EDGE('',*,*,#48905,.T.);
#64954=ORIENTED_EDGE('',*,*,#48906,.T.);
#64955=ORIENTED_EDGE('',*,*,#48907,.T.);
#64956=ORIENTED_EDGE('',*,*,#48908,.T.);
#64957=ORIENTED_EDGE('',*,*,#48909,.T.);
#64958=ORIENTED_EDGE('',*,*,#48910,.T.);
#64959=ORIENTED_EDGE('',*,*,#48911,.T.);
#64960=ORIENTED_EDGE('',*,*,#48912,.T.);
#64961=ORIENTED_EDGE('',*,*,#48913,.T.);
#64962=ORIENTED_EDGE('',*,*,#48914,.T.);
#64963=ORIENTED_EDGE('',*,*,#48915,.T.);
#64964=ORIENTED_EDGE('',*,*,#48916,.T.);
#64965=ORIENTED_EDGE('',*,*,#48917,.T.);
#64966=ORIENTED_EDGE('',*,*,#48918,.T.);
#64967=ORIENTED_EDGE('',*,*,#48919,.T.);
#64968=ORIENTED_EDGE('',*,*,#48920,.T.);
#64969=ORIENTED_EDGE('',*,*,#48921,.T.);
#64970=ORIENTED_EDGE('',*,*,#48922,.T.);
#64971=ORIENTED_EDGE('',*,*,#48923,.T.);
#64972=ORIENTED_EDGE('',*,*,#48924,.T.);
#64973=ORIENTED_EDGE('',*,*,#48925,.T.);
#64974=ORIENTED_EDGE('',*,*,#48926,.T.);
#64975=ORIENTED_EDGE('',*,*,#48927,.T.);
#64976=ORIENTED_EDGE('',*,*,#48928,.T.);
#64977=ORIENTED_EDGE('',*,*,#48929,.T.);
#64978=ORIENTED_EDGE('',*,*,#48930,.T.);
#64979=ORIENTED_EDGE('',*,*,#48931,.T.);
#64980=ORIENTED_EDGE('',*,*,#48932,.T.);
#64981=ORIENTED_EDGE('',*,*,#48933,.T.);
#64982=ORIENTED_EDGE('',*,*,#48934,.T.);
#64983=ORIENTED_EDGE('',*,*,#48935,.T.);
#64984=ORIENTED_EDGE('',*,*,#48936,.T.);
#64985=ORIENTED_EDGE('',*,*,#48937,.T.);
#64986=ORIENTED_EDGE('',*,*,#48938,.T.);
#64987=ORIENTED_EDGE('',*,*,#48939,.T.);
#64988=ORIENTED_EDGE('',*,*,#48940,.T.);
#64989=ORIENTED_EDGE('',*,*,#48941,.T.);
#64990=ORIENTED_EDGE('',*,*,#48942,.T.);
#64991=ORIENTED_EDGE('',*,*,#48943,.T.);
#64992=ORIENTED_EDGE('',*,*,#48944,.T.);
#64993=ORIENTED_EDGE('',*,*,#48945,.T.);
#64994=ORIENTED_EDGE('',*,*,#48946,.T.);
#64995=ORIENTED_EDGE('',*,*,#48947,.T.);
#64996=ORIENTED_EDGE('',*,*,#48948,.T.);
#64997=ORIENTED_EDGE('',*,*,#48949,.T.);
#64998=ORIENTED_EDGE('',*,*,#48950,.T.);
#64999=ORIENTED_EDGE('',*,*,#48951,.T.);
#65000=ORIENTED_EDGE('',*,*,#48952,.T.);
#65001=ORIENTED_EDGE('',*,*,#48953,.T.);
#65002=ORIENTED_EDGE('',*,*,#48954,.T.);
#65003=ORIENTED_EDGE('',*,*,#48955,.T.);
#65004=ORIENTED_EDGE('',*,*,#48956,.T.);
#65005=ORIENTED_EDGE('',*,*,#48957,.T.);
#65006=ORIENTED_EDGE('',*,*,#48958,.T.);
#65007=ORIENTED_EDGE('',*,*,#48959,.T.);
#65008=ORIENTED_EDGE('',*,*,#48960,.T.);
#65009=ORIENTED_EDGE('',*,*,#48961,.T.);
#65010=ORIENTED_EDGE('',*,*,#48962,.T.);
#65011=ORIENTED_EDGE('',*,*,#48963,.T.);
#65012=ORIENTED_EDGE('',*,*,#48964,.T.);
#65013=ORIENTED_EDGE('',*,*,#48965,.T.);
#65014=ORIENTED_EDGE('',*,*,#48966,.T.);
#65015=ORIENTED_EDGE('',*,*,#48967,.T.);
#65016=ORIENTED_EDGE('',*,*,#48968,.T.);
#65017=ORIENTED_EDGE('',*,*,#48969,.T.);
#65018=ORIENTED_EDGE('',*,*,#48970,.T.);
#65019=ORIENTED_EDGE('',*,*,#48971,.T.);
#65020=ORIENTED_EDGE('',*,*,#48972,.T.);
#65021=ORIENTED_EDGE('',*,*,#48973,.T.);
#65022=ORIENTED_EDGE('',*,*,#48974,.T.);
#65023=ORIENTED_EDGE('',*,*,#48975,.T.);
#65024=ORIENTED_EDGE('',*,*,#48976,.T.);
#65025=ORIENTED_EDGE('',*,*,#48977,.T.);
#65026=ORIENTED_EDGE('',*,*,#48978,.T.);
#65027=ORIENTED_EDGE('',*,*,#48979,.T.);
#65028=ORIENTED_EDGE('',*,*,#48980,.T.);
#65029=ORIENTED_EDGE('',*,*,#48981,.T.);
#65030=ORIENTED_EDGE('',*,*,#48982,.T.);
#65031=ORIENTED_EDGE('',*,*,#48983,.T.);
#65032=ORIENTED_EDGE('',*,*,#48984,.T.);
#65033=ORIENTED_EDGE('',*,*,#48985,.T.);
#65034=ORIENTED_EDGE('',*,*,#48986,.T.);
#65035=ORIENTED_EDGE('',*,*,#48987,.T.);
#65036=ORIENTED_EDGE('',*,*,#48988,.T.);
#65037=ORIENTED_EDGE('',*,*,#48989,.T.);
#65038=ORIENTED_EDGE('',*,*,#48990,.T.);
#65039=ORIENTED_EDGE('',*,*,#48991,.T.);
#65040=ORIENTED_EDGE('',*,*,#48992,.T.);
#65041=ORIENTED_EDGE('',*,*,#48993,.T.);
#65042=ORIENTED_EDGE('',*,*,#48994,.T.);
#65043=ORIENTED_EDGE('',*,*,#48995,.T.);
#65044=ORIENTED_EDGE('',*,*,#48996,.T.);
#65045=ORIENTED_EDGE('',*,*,#48997,.T.);
#65046=ORIENTED_EDGE('',*,*,#48998,.T.);
#65047=ORIENTED_EDGE('',*,*,#48999,.T.);
#65048=ORIENTED_EDGE('',*,*,#49000,.T.);
#65049=ORIENTED_EDGE('',*,*,#49001,.T.);
#65050=ORIENTED_EDGE('',*,*,#49002,.T.);
#65051=ORIENTED_EDGE('',*,*,#49003,.T.);
#65052=ORIENTED_EDGE('',*,*,#49004,.T.);
#65053=ORIENTED_EDGE('',*,*,#49005,.T.);
#65054=ORIENTED_EDGE('',*,*,#49006,.T.);
#65055=ORIENTED_EDGE('',*,*,#49007,.T.);
#65056=ORIENTED_EDGE('',*,*,#49008,.T.);
#65057=ORIENTED_EDGE('',*,*,#49009,.T.);
#65058=ORIENTED_EDGE('',*,*,#49010,.T.);
#65059=ORIENTED_EDGE('',*,*,#49011,.T.);
#65060=ORIENTED_EDGE('',*,*,#49012,.T.);
#65061=ORIENTED_EDGE('',*,*,#49013,.T.);
#65062=ORIENTED_EDGE('',*,*,#49014,.T.);
#65063=ORIENTED_EDGE('',*,*,#49015,.T.);
#65064=ORIENTED_EDGE('',*,*,#49016,.T.);
#65065=ORIENTED_EDGE('',*,*,#49017,.T.);
#65066=ORIENTED_EDGE('',*,*,#49018,.T.);
#65067=ORIENTED_EDGE('',*,*,#49019,.T.);
#65068=ORIENTED_EDGE('',*,*,#49020,.T.);
#65069=ORIENTED_EDGE('',*,*,#49021,.T.);
#65070=ORIENTED_EDGE('',*,*,#49022,.T.);
#65071=ORIENTED_EDGE('',*,*,#49023,.T.);
#65072=ORIENTED_EDGE('',*,*,#49024,.T.);
#65073=ORIENTED_EDGE('',*,*,#49025,.T.);
#65074=ORIENTED_EDGE('',*,*,#49026,.T.);
#65075=ORIENTED_EDGE('',*,*,#49027,.T.);
#65076=ORIENTED_EDGE('',*,*,#49028,.T.);
#65077=ORIENTED_EDGE('',*,*,#49029,.T.);
#65078=ORIENTED_EDGE('',*,*,#49030,.T.);
#65079=ORIENTED_EDGE('',*,*,#49031,.T.);
#65080=ORIENTED_EDGE('',*,*,#49032,.T.);
#65081=ORIENTED_EDGE('',*,*,#49033,.T.);
#65082=ORIENTED_EDGE('',*,*,#49034,.T.);
#65083=ORIENTED_EDGE('',*,*,#49035,.T.);
#65084=ORIENTED_EDGE('',*,*,#49036,.T.);
#65085=ORIENTED_EDGE('',*,*,#49037,.T.);
#65086=ORIENTED_EDGE('',*,*,#49038,.T.);
#65087=ORIENTED_EDGE('',*,*,#49039,.T.);
#65088=ORIENTED_EDGE('',*,*,#49040,.T.);
#65089=ORIENTED_EDGE('',*,*,#49041,.T.);
#65090=ORIENTED_EDGE('',*,*,#49042,.T.);
#65091=ORIENTED_EDGE('',*,*,#49043,.T.);
#65092=ORIENTED_EDGE('',*,*,#49044,.T.);
#65093=ORIENTED_EDGE('',*,*,#49045,.T.);
#65094=ORIENTED_EDGE('',*,*,#49046,.T.);
#65095=ORIENTED_EDGE('',*,*,#49047,.T.);
#65096=ORIENTED_EDGE('',*,*,#49048,.T.);
#65097=ORIENTED_EDGE('',*,*,#49049,.T.);
#65098=ORIENTED_EDGE('',*,*,#49050,.T.);
#65099=ORIENTED_EDGE('',*,*,#49051,.T.);
#65100=ORIENTED_EDGE('',*,*,#49052,.T.);
#65101=ORIENTED_EDGE('',*,*,#49053,.T.);
#65102=ORIENTED_EDGE('',*,*,#49054,.T.);
#65103=ORIENTED_EDGE('',*,*,#49055,.T.);
#65104=ORIENTED_EDGE('',*,*,#49056,.T.);
#65105=ORIENTED_EDGE('',*,*,#49057,.T.);
#65106=ORIENTED_EDGE('',*,*,#49058,.T.);
#65107=ORIENTED_EDGE('',*,*,#49059,.T.);
#65108=ORIENTED_EDGE('',*,*,#49060,.T.);
#65109=ORIENTED_EDGE('',*,*,#49061,.T.);
#65110=ORIENTED_EDGE('',*,*,#49062,.T.);
#65111=ORIENTED_EDGE('',*,*,#49063,.T.);
#65112=ORIENTED_EDGE('',*,*,#49064,.T.);
#65113=ORIENTED_EDGE('',*,*,#49065,.T.);
#65114=ORIENTED_EDGE('',*,*,#49066,.T.);
#65115=ORIENTED_EDGE('',*,*,#49067,.T.);
#65116=ORIENTED_EDGE('',*,*,#49068,.T.);
#65117=ORIENTED_EDGE('',*,*,#49069,.T.);
#65118=ORIENTED_EDGE('',*,*,#49070,.T.);
#65119=ORIENTED_EDGE('',*,*,#49071,.T.);
#65120=ORIENTED_EDGE('',*,*,#49072,.T.);
#65121=ORIENTED_EDGE('',*,*,#49073,.T.);
#65122=ORIENTED_EDGE('',*,*,#49074,.T.);
#65123=ORIENTED_EDGE('',*,*,#49075,.T.);
#65124=ORIENTED_EDGE('',*,*,#49076,.T.);
#65125=ORIENTED_EDGE('',*,*,#49077,.T.);
#65126=ORIENTED_EDGE('',*,*,#49078,.T.);
#65127=ORIENTED_EDGE('',*,*,#49079,.T.);
#65128=ORIENTED_EDGE('',*,*,#49080,.T.);
#65129=ORIENTED_EDGE('',*,*,#49081,.T.);
#65130=ORIENTED_EDGE('',*,*,#49082,.T.);
#65131=ORIENTED_EDGE('',*,*,#49083,.T.);
#65132=ORIENTED_EDGE('',*,*,#49084,.T.);
#65133=ORIENTED_EDGE('',*,*,#49085,.T.);
#65134=ORIENTED_EDGE('',*,*,#49086,.T.);
#65135=ORIENTED_EDGE('',*,*,#49087,.T.);
#65136=ORIENTED_EDGE('',*,*,#49088,.T.);
#65137=ORIENTED_EDGE('',*,*,#49089,.T.);
#65138=ORIENTED_EDGE('',*,*,#49090,.T.);
#65139=ORIENTED_EDGE('',*,*,#49091,.T.);
#65140=ORIENTED_EDGE('',*,*,#49092,.T.);
#65141=ORIENTED_EDGE('',*,*,#49093,.T.);
#65142=ORIENTED_EDGE('',*,*,#49094,.T.);
#65143=ORIENTED_EDGE('',*,*,#49095,.T.);
#65144=ORIENTED_EDGE('',*,*,#49096,.T.);
#65145=ORIENTED_EDGE('',*,*,#49097,.T.);
#65146=ORIENTED_EDGE('',*,*,#49098,.T.);
#65147=ORIENTED_EDGE('',*,*,#49099,.T.);
#65148=ORIENTED_EDGE('',*,*,#49100,.T.);
#65149=ORIENTED_EDGE('',*,*,#49101,.T.);
#65150=ORIENTED_EDGE('',*,*,#49102,.T.);
#65151=ORIENTED_EDGE('',*,*,#49103,.T.);
#65152=ORIENTED_EDGE('',*,*,#49104,.T.);
#65153=ORIENTED_EDGE('',*,*,#49105,.T.);
#65154=ORIENTED_EDGE('',*,*,#49106,.T.);
#65155=ORIENTED_EDGE('',*,*,#49107,.T.);
#65156=ORIENTED_EDGE('',*,*,#49108,.T.);
#65157=ORIENTED_EDGE('',*,*,#49109,.T.);
#65158=ORIENTED_EDGE('',*,*,#49110,.T.);
#65159=ORIENTED_EDGE('',*,*,#49111,.T.);
#65160=ORIENTED_EDGE('',*,*,#49112,.T.);
#65161=ORIENTED_EDGE('',*,*,#49113,.T.);
#65162=ORIENTED_EDGE('',*,*,#49114,.T.);
#65163=ORIENTED_EDGE('',*,*,#49115,.T.);
#65164=ORIENTED_EDGE('',*,*,#49116,.T.);
#65165=ORIENTED_EDGE('',*,*,#49117,.T.);
#65166=ORIENTED_EDGE('',*,*,#49118,.T.);
#65167=ORIENTED_EDGE('',*,*,#49119,.T.);
#65168=ORIENTED_EDGE('',*,*,#49120,.T.);
#65169=ORIENTED_EDGE('',*,*,#49121,.T.);
#65170=ORIENTED_EDGE('',*,*,#49122,.T.);
#65171=ORIENTED_EDGE('',*,*,#49123,.T.);
#65172=ORIENTED_EDGE('',*,*,#49124,.T.);
#65173=ORIENTED_EDGE('',*,*,#49125,.T.);
#65174=ORIENTED_EDGE('',*,*,#49126,.T.);
#65175=ORIENTED_EDGE('',*,*,#49127,.T.);
#65176=ORIENTED_EDGE('',*,*,#49128,.T.);
#65177=ORIENTED_EDGE('',*,*,#49129,.T.);
#65178=ORIENTED_EDGE('',*,*,#49130,.T.);
#65179=ORIENTED_EDGE('',*,*,#49131,.T.);
#65180=ORIENTED_EDGE('',*,*,#49132,.T.);
#65181=ORIENTED_EDGE('',*,*,#49133,.T.);
#65182=ORIENTED_EDGE('',*,*,#49134,.T.);
#65183=ORIENTED_EDGE('',*,*,#49135,.T.);
#65184=ORIENTED_EDGE('',*,*,#49136,.T.);
#65185=ORIENTED_EDGE('',*,*,#49137,.T.);
#65186=ORIENTED_EDGE('',*,*,#49138,.T.);
#65187=ORIENTED_EDGE('',*,*,#49139,.T.);
#65188=ORIENTED_EDGE('',*,*,#49140,.T.);
#65189=ORIENTED_EDGE('',*,*,#49141,.T.);
#65190=ORIENTED_EDGE('',*,*,#49142,.T.);
#65191=ORIENTED_EDGE('',*,*,#49143,.T.);
#65192=ORIENTED_EDGE('',*,*,#49144,.T.);
#65193=ORIENTED_EDGE('',*,*,#49145,.T.);
#65194=ORIENTED_EDGE('',*,*,#49146,.T.);
#65195=ORIENTED_EDGE('',*,*,#49147,.T.);
#65196=ORIENTED_EDGE('',*,*,#49148,.T.);
#65197=ORIENTED_EDGE('',*,*,#49149,.T.);
#65198=ORIENTED_EDGE('',*,*,#49150,.T.);
#65199=ORIENTED_EDGE('',*,*,#49151,.T.);
#65200=ORIENTED_EDGE('',*,*,#49152,.T.);
#65201=ORIENTED_EDGE('',*,*,#49153,.T.);
#65202=ORIENTED_EDGE('',*,*,#49154,.T.);
#65203=ORIENTED_EDGE('',*,*,#49155,.T.);
#65204=ORIENTED_EDGE('',*,*,#49156,.T.);
#65205=ORIENTED_EDGE('',*,*,#49157,.T.);
#65206=ORIENTED_EDGE('',*,*,#49158,.T.);
#65207=ORIENTED_EDGE('',*,*,#49159,.T.);
#65208=ORIENTED_EDGE('',*,*,#49160,.T.);
#65209=ORIENTED_EDGE('',*,*,#49161,.T.);
#65210=ORIENTED_EDGE('',*,*,#49162,.T.);
#65211=ORIENTED_EDGE('',*,*,#49163,.T.);
#65212=ORIENTED_EDGE('',*,*,#49164,.T.);
#65213=ORIENTED_EDGE('',*,*,#49165,.T.);
#65214=ORIENTED_EDGE('',*,*,#49166,.T.);
#65215=ORIENTED_EDGE('',*,*,#49167,.T.);
#65216=ORIENTED_EDGE('',*,*,#49168,.T.);
#65217=ORIENTED_EDGE('',*,*,#49169,.T.);
#65218=ORIENTED_EDGE('',*,*,#49170,.T.);
#65219=ORIENTED_EDGE('',*,*,#49171,.T.);
#65220=ORIENTED_EDGE('',*,*,#49172,.T.);
#65221=ORIENTED_EDGE('',*,*,#49173,.T.);
#65222=ORIENTED_EDGE('',*,*,#49174,.T.);
#65223=ORIENTED_EDGE('',*,*,#49175,.T.);
#65224=ORIENTED_EDGE('',*,*,#49176,.T.);
#65225=ORIENTED_EDGE('',*,*,#49177,.T.);
#65226=ORIENTED_EDGE('',*,*,#49178,.T.);
#65227=ORIENTED_EDGE('',*,*,#49179,.T.);
#65228=ORIENTED_EDGE('',*,*,#49180,.T.);
#65229=ORIENTED_EDGE('',*,*,#49181,.T.);
#65230=ORIENTED_EDGE('',*,*,#49182,.T.);
#65231=ORIENTED_EDGE('',*,*,#49183,.T.);
#65232=ORIENTED_EDGE('',*,*,#49184,.T.);
#65233=ORIENTED_EDGE('',*,*,#49185,.T.);
#65234=ORIENTED_EDGE('',*,*,#49186,.T.);
#65235=ORIENTED_EDGE('',*,*,#49187,.T.);
#65236=ORIENTED_EDGE('',*,*,#49188,.T.);
#65237=ORIENTED_EDGE('',*,*,#49189,.T.);
#65238=ORIENTED_EDGE('',*,*,#49190,.T.);
#65239=ORIENTED_EDGE('',*,*,#49191,.T.);
#65240=ORIENTED_EDGE('',*,*,#49192,.T.);
#65241=ORIENTED_EDGE('',*,*,#49193,.T.);
#65242=ORIENTED_EDGE('',*,*,#49194,.T.);
#65243=ORIENTED_EDGE('',*,*,#49195,.T.);
#65244=ORIENTED_EDGE('',*,*,#49196,.T.);
#65245=ORIENTED_EDGE('',*,*,#49197,.T.);
#65246=ORIENTED_EDGE('',*,*,#49198,.T.);
#65247=ORIENTED_EDGE('',*,*,#49199,.T.);
#65248=ORIENTED_EDGE('',*,*,#49200,.T.);
#65249=ORIENTED_EDGE('',*,*,#49201,.T.);
#65250=ORIENTED_EDGE('',*,*,#49202,.T.);
#65251=ORIENTED_EDGE('',*,*,#49203,.T.);
#65252=ORIENTED_EDGE('',*,*,#49204,.T.);
#65253=ORIENTED_EDGE('',*,*,#49205,.T.);
#65254=ORIENTED_EDGE('',*,*,#49206,.T.);
#65255=ORIENTED_EDGE('',*,*,#49207,.T.);
#65256=ORIENTED_EDGE('',*,*,#49208,.T.);
#65257=ORIENTED_EDGE('',*,*,#49209,.T.);
#65258=ORIENTED_EDGE('',*,*,#49210,.T.);
#65259=ORIENTED_EDGE('',*,*,#49211,.T.);
#65260=ORIENTED_EDGE('',*,*,#49212,.T.);
#65261=ORIENTED_EDGE('',*,*,#49213,.T.);
#65262=ORIENTED_EDGE('',*,*,#49214,.T.);
#65263=ORIENTED_EDGE('',*,*,#49215,.T.);
#65264=ORIENTED_EDGE('',*,*,#49216,.T.);
#65265=ORIENTED_EDGE('',*,*,#49217,.T.);
#65266=ORIENTED_EDGE('',*,*,#49218,.T.);
#65267=ORIENTED_EDGE('',*,*,#49219,.T.);
#65268=ORIENTED_EDGE('',*,*,#49220,.T.);
#65269=ORIENTED_EDGE('',*,*,#49221,.T.);
#65270=ORIENTED_EDGE('',*,*,#49222,.T.);
#65271=ORIENTED_EDGE('',*,*,#49223,.T.);
#65272=ORIENTED_EDGE('',*,*,#49224,.T.);
#65273=ORIENTED_EDGE('',*,*,#49225,.T.);
#65274=ORIENTED_EDGE('',*,*,#49226,.T.);
#65275=ORIENTED_EDGE('',*,*,#49227,.T.);
#65276=ORIENTED_EDGE('',*,*,#49228,.T.);
#65277=ORIENTED_EDGE('',*,*,#49229,.T.);
#65278=ORIENTED_EDGE('',*,*,#49230,.T.);
#65279=ORIENTED_EDGE('',*,*,#49231,.T.);
#65280=ORIENTED_EDGE('',*,*,#49232,.T.);
#65281=ORIENTED_EDGE('',*,*,#49233,.T.);
#65282=ORIENTED_EDGE('',*,*,#49234,.T.);
#65283=ORIENTED_EDGE('',*,*,#49235,.T.);
#65284=ORIENTED_EDGE('',*,*,#49236,.T.);
#65285=ORIENTED_EDGE('',*,*,#49237,.T.);
#65286=ORIENTED_EDGE('',*,*,#49238,.T.);
#65287=ORIENTED_EDGE('',*,*,#49239,.T.);
#65288=ORIENTED_EDGE('',*,*,#49240,.T.);
#65289=ORIENTED_EDGE('',*,*,#49241,.T.);
#65290=ORIENTED_EDGE('',*,*,#49242,.T.);
#65291=ORIENTED_EDGE('',*,*,#49243,.T.);
#65292=ORIENTED_EDGE('',*,*,#49244,.T.);
#65293=ORIENTED_EDGE('',*,*,#49245,.T.);
#65294=ORIENTED_EDGE('',*,*,#49246,.T.);
#65295=ORIENTED_EDGE('',*,*,#49247,.T.);
#65296=ORIENTED_EDGE('',*,*,#49248,.T.);
#65297=ORIENTED_EDGE('',*,*,#49249,.T.);
#65298=ORIENTED_EDGE('',*,*,#49250,.T.);
#65299=ORIENTED_EDGE('',*,*,#49251,.T.);
#65300=ORIENTED_EDGE('',*,*,#49252,.T.);
#65301=ORIENTED_EDGE('',*,*,#49253,.T.);
#65302=ORIENTED_EDGE('',*,*,#49254,.T.);
#65303=ORIENTED_EDGE('',*,*,#49255,.T.);
#65304=ORIENTED_EDGE('',*,*,#49256,.T.);
#65305=ORIENTED_EDGE('',*,*,#49257,.T.);
#65306=ORIENTED_EDGE('',*,*,#49258,.T.);
#65307=ORIENTED_EDGE('',*,*,#49259,.T.);
#65308=ORIENTED_EDGE('',*,*,#49260,.T.);
#65309=ORIENTED_EDGE('',*,*,#49261,.T.);
#65310=ORIENTED_EDGE('',*,*,#49262,.T.);
#65311=ORIENTED_EDGE('',*,*,#49263,.T.);
#65312=ORIENTED_EDGE('',*,*,#49264,.T.);
#65313=ORIENTED_EDGE('',*,*,#49265,.T.);
#65314=ORIENTED_EDGE('',*,*,#49266,.T.);
#65315=ORIENTED_EDGE('',*,*,#49267,.T.);
#65316=ORIENTED_EDGE('',*,*,#49268,.T.);
#65317=ORIENTED_EDGE('',*,*,#49269,.T.);
#65318=ORIENTED_EDGE('',*,*,#49270,.T.);
#65319=ORIENTED_EDGE('',*,*,#49271,.T.);
#65320=ORIENTED_EDGE('',*,*,#49272,.T.);
#65321=ORIENTED_EDGE('',*,*,#49273,.T.);
#65322=ORIENTED_EDGE('',*,*,#49274,.T.);
#65323=ORIENTED_EDGE('',*,*,#49275,.T.);
#65324=ORIENTED_EDGE('',*,*,#49276,.T.);
#65325=ORIENTED_EDGE('',*,*,#49277,.T.);
#65326=ORIENTED_EDGE('',*,*,#49278,.T.);
#65327=ORIENTED_EDGE('',*,*,#49279,.T.);
#65328=ORIENTED_EDGE('',*,*,#49280,.T.);
#65329=ORIENTED_EDGE('',*,*,#49281,.T.);
#65330=ORIENTED_EDGE('',*,*,#49282,.T.);
#65331=ORIENTED_EDGE('',*,*,#49283,.T.);
#65332=ORIENTED_EDGE('',*,*,#49284,.T.);
#65333=ORIENTED_EDGE('',*,*,#49285,.T.);
#65334=ORIENTED_EDGE('',*,*,#49286,.T.);
#65335=ORIENTED_EDGE('',*,*,#49287,.T.);
#65336=ORIENTED_EDGE('',*,*,#49288,.T.);
#65337=ORIENTED_EDGE('',*,*,#49289,.T.);
#65338=ORIENTED_EDGE('',*,*,#49290,.T.);
#65339=ORIENTED_EDGE('',*,*,#49291,.T.);
#65340=ORIENTED_EDGE('',*,*,#49292,.T.);
#65341=ORIENTED_EDGE('',*,*,#49293,.T.);
#65342=ORIENTED_EDGE('',*,*,#49294,.T.);
#65343=ORIENTED_EDGE('',*,*,#49295,.T.);
#65344=ORIENTED_EDGE('',*,*,#49296,.T.);
#65345=ORIENTED_EDGE('',*,*,#49297,.T.);
#65346=ORIENTED_EDGE('',*,*,#49298,.T.);
#65347=ORIENTED_EDGE('',*,*,#49299,.T.);
#65348=ORIENTED_EDGE('',*,*,#49300,.T.);
#65349=ORIENTED_EDGE('',*,*,#49301,.T.);
#65350=ORIENTED_EDGE('',*,*,#49302,.T.);
#65351=ORIENTED_EDGE('',*,*,#49303,.T.);
#65352=ORIENTED_EDGE('',*,*,#49304,.T.);
#65353=ORIENTED_EDGE('',*,*,#49305,.T.);
#65354=ORIENTED_EDGE('',*,*,#49306,.T.);
#65355=ORIENTED_EDGE('',*,*,#49307,.T.);
#65356=ORIENTED_EDGE('',*,*,#49308,.T.);
#65357=ORIENTED_EDGE('',*,*,#49309,.T.);
#65358=ORIENTED_EDGE('',*,*,#49310,.T.);
#65359=ORIENTED_EDGE('',*,*,#49311,.T.);
#65360=ORIENTED_EDGE('',*,*,#49312,.T.);
#65361=ORIENTED_EDGE('',*,*,#49313,.T.);
#65362=ORIENTED_EDGE('',*,*,#45896,.T.);
#65363=ORIENTED_EDGE('',*,*,#49314,.T.);
#65364=ORIENTED_EDGE('',*,*,#45890,.T.);
#65365=ORIENTED_EDGE('',*,*,#49315,.T.);
#65366=ORIENTED_EDGE('',*,*,#49316,.T.);
#65367=ORIENTED_EDGE('',*,*,#49317,.T.);
#65368=ORIENTED_EDGE('',*,*,#49318,.T.);
#65369=ORIENTED_EDGE('',*,*,#49319,.T.);
#65370=ORIENTED_EDGE('',*,*,#49320,.T.);
#65371=ORIENTED_EDGE('',*,*,#49321,.T.);
#65372=ORIENTED_EDGE('',*,*,#49322,.T.);
#65373=ORIENTED_EDGE('',*,*,#49323,.T.);
#65374=ORIENTED_EDGE('',*,*,#49324,.T.);
#65375=ORIENTED_EDGE('',*,*,#49325,.T.);
#65376=ORIENTED_EDGE('',*,*,#49326,.T.);
#65377=ORIENTED_EDGE('',*,*,#49327,.T.);
#65378=ORIENTED_EDGE('',*,*,#49328,.T.);
#65379=ORIENTED_EDGE('',*,*,#49329,.T.);
#65380=ORIENTED_EDGE('',*,*,#49330,.T.);
#65381=ORIENTED_EDGE('',*,*,#49331,.T.);
#65382=ORIENTED_EDGE('',*,*,#49332,.T.);
#65383=ORIENTED_EDGE('',*,*,#49333,.T.);
#65384=ORIENTED_EDGE('',*,*,#49334,.T.);
#65385=ORIENTED_EDGE('',*,*,#49335,.T.);
#65386=ORIENTED_EDGE('',*,*,#49336,.T.);
#65387=ORIENTED_EDGE('',*,*,#49337,.T.);
#65388=ORIENTED_EDGE('',*,*,#49338,.T.);
#65389=ORIENTED_EDGE('',*,*,#49339,.T.);
#65390=ORIENTED_EDGE('',*,*,#49340,.T.);
#65391=ORIENTED_EDGE('',*,*,#49341,.T.);
#65392=ORIENTED_EDGE('',*,*,#49342,.T.);
#65393=ORIENTED_EDGE('',*,*,#49343,.T.);
#65394=ORIENTED_EDGE('',*,*,#49344,.T.);
#65395=ORIENTED_EDGE('',*,*,#49345,.T.);
#65396=ORIENTED_EDGE('',*,*,#49346,.T.);
#65397=ORIENTED_EDGE('',*,*,#49347,.T.);
#65398=ORIENTED_EDGE('',*,*,#49348,.T.);
#65399=ORIENTED_EDGE('',*,*,#49349,.T.);
#65400=ORIENTED_EDGE('',*,*,#49350,.T.);
#65401=ORIENTED_EDGE('',*,*,#49351,.T.);
#65402=ORIENTED_EDGE('',*,*,#49352,.T.);
#65403=ORIENTED_EDGE('',*,*,#49353,.T.);
#65404=ORIENTED_EDGE('',*,*,#49354,.T.);
#65405=ORIENTED_EDGE('',*,*,#49355,.T.);
#65406=ORIENTED_EDGE('',*,*,#49356,.T.);
#65407=ORIENTED_EDGE('',*,*,#49357,.T.);
#65408=ORIENTED_EDGE('',*,*,#49358,.T.);
#65409=ORIENTED_EDGE('',*,*,#49359,.T.);
#65410=ORIENTED_EDGE('',*,*,#49360,.T.);
#65411=ORIENTED_EDGE('',*,*,#49361,.T.);
#65412=ORIENTED_EDGE('',*,*,#49362,.T.);
#65413=ORIENTED_EDGE('',*,*,#49363,.T.);
#65414=ORIENTED_EDGE('',*,*,#49364,.T.);
#65415=ORIENTED_EDGE('',*,*,#49365,.T.);
#65416=ORIENTED_EDGE('',*,*,#49366,.T.);
#65417=ORIENTED_EDGE('',*,*,#49367,.T.);
#65418=ORIENTED_EDGE('',*,*,#49368,.T.);
#65419=ORIENTED_EDGE('',*,*,#49369,.T.);
#65420=ORIENTED_EDGE('',*,*,#49370,.T.);
#65421=ORIENTED_EDGE('',*,*,#49371,.T.);
#65422=ORIENTED_EDGE('',*,*,#49372,.T.);
#65423=ORIENTED_EDGE('',*,*,#49373,.T.);
#65424=ORIENTED_EDGE('',*,*,#49374,.T.);
#65425=ORIENTED_EDGE('',*,*,#49375,.T.);
#65426=ORIENTED_EDGE('',*,*,#49376,.T.);
#65427=ORIENTED_EDGE('',*,*,#49377,.T.);
#65428=ORIENTED_EDGE('',*,*,#49378,.T.);
#65429=ORIENTED_EDGE('',*,*,#49379,.T.);
#65430=ORIENTED_EDGE('',*,*,#49380,.T.);
#65431=ORIENTED_EDGE('',*,*,#49381,.T.);
#65432=ORIENTED_EDGE('',*,*,#49382,.T.);
#65433=ORIENTED_EDGE('',*,*,#49383,.T.);
#65434=ORIENTED_EDGE('',*,*,#49384,.T.);
#65435=ORIENTED_EDGE('',*,*,#49385,.T.);
#65436=ORIENTED_EDGE('',*,*,#49386,.T.);
#65437=ORIENTED_EDGE('',*,*,#49387,.T.);
#65438=ORIENTED_EDGE('',*,*,#49388,.T.);
#65439=ORIENTED_EDGE('',*,*,#49389,.T.);
#65440=ORIENTED_EDGE('',*,*,#49390,.T.);
#65441=ORIENTED_EDGE('',*,*,#49391,.T.);
#65442=ORIENTED_EDGE('',*,*,#49392,.T.);
#65443=ORIENTED_EDGE('',*,*,#49393,.T.);
#65444=ORIENTED_EDGE('',*,*,#49394,.T.);
#65445=ORIENTED_EDGE('',*,*,#49395,.T.);
#65446=ORIENTED_EDGE('',*,*,#49396,.T.);
#65447=ORIENTED_EDGE('',*,*,#49397,.T.);
#65448=ORIENTED_EDGE('',*,*,#49398,.T.);
#65449=ORIENTED_EDGE('',*,*,#49399,.T.);
#65450=ORIENTED_EDGE('',*,*,#49400,.T.);
#65451=ORIENTED_EDGE('',*,*,#49401,.T.);
#65452=ORIENTED_EDGE('',*,*,#49402,.T.);
#65453=ORIENTED_EDGE('',*,*,#49403,.T.);
#65454=ORIENTED_EDGE('',*,*,#49404,.T.);
#65455=ORIENTED_EDGE('',*,*,#49405,.T.);
#65456=ORIENTED_EDGE('',*,*,#49406,.T.);
#65457=ORIENTED_EDGE('',*,*,#49407,.T.);
#65458=ORIENTED_EDGE('',*,*,#49408,.T.);
#65459=ORIENTED_EDGE('',*,*,#49409,.T.);
#65460=ORIENTED_EDGE('',*,*,#49410,.T.);
#65461=ORIENTED_EDGE('',*,*,#49411,.T.);
#65462=ORIENTED_EDGE('',*,*,#49412,.T.);
#65463=ORIENTED_EDGE('',*,*,#49413,.T.);
#65464=ORIENTED_EDGE('',*,*,#49414,.T.);
#65465=ORIENTED_EDGE('',*,*,#49415,.T.);
#65466=ORIENTED_EDGE('',*,*,#49416,.T.);
#65467=ORIENTED_EDGE('',*,*,#49417,.T.);
#65468=ORIENTED_EDGE('',*,*,#49418,.T.);
#65469=ORIENTED_EDGE('',*,*,#49419,.T.);
#65470=ORIENTED_EDGE('',*,*,#49420,.T.);
#65471=ORIENTED_EDGE('',*,*,#49421,.T.);
#65472=ORIENTED_EDGE('',*,*,#49422,.T.);
#65473=ORIENTED_EDGE('',*,*,#49423,.T.);
#65474=ORIENTED_EDGE('',*,*,#49424,.T.);
#65475=ORIENTED_EDGE('',*,*,#49425,.T.);
#65476=ORIENTED_EDGE('',*,*,#49426,.T.);
#65477=ORIENTED_EDGE('',*,*,#49427,.T.);
#65478=ORIENTED_EDGE('',*,*,#49428,.T.);
#65479=ORIENTED_EDGE('',*,*,#49429,.T.);
#65480=ORIENTED_EDGE('',*,*,#49430,.T.);
#65481=ORIENTED_EDGE('',*,*,#49431,.T.);
#65482=ORIENTED_EDGE('',*,*,#49432,.T.);
#65483=ORIENTED_EDGE('',*,*,#49433,.T.);
#65484=ORIENTED_EDGE('',*,*,#49434,.T.);
#65485=ORIENTED_EDGE('',*,*,#49435,.T.);
#65486=ORIENTED_EDGE('',*,*,#49436,.T.);
#65487=ORIENTED_EDGE('',*,*,#49437,.T.);
#65488=ORIENTED_EDGE('',*,*,#49438,.T.);
#65489=ORIENTED_EDGE('',*,*,#49439,.T.);
#65490=ORIENTED_EDGE('',*,*,#49440,.T.);
#65491=ORIENTED_EDGE('',*,*,#49441,.T.);
#65492=ORIENTED_EDGE('',*,*,#49442,.T.);
#65493=ORIENTED_EDGE('',*,*,#49443,.T.);
#65494=ORIENTED_EDGE('',*,*,#49444,.T.);
#65495=ORIENTED_EDGE('',*,*,#49445,.T.);
#65496=ORIENTED_EDGE('',*,*,#49446,.T.);
#65497=ORIENTED_EDGE('',*,*,#49447,.T.);
#65498=ORIENTED_EDGE('',*,*,#49448,.T.);
#65499=ORIENTED_EDGE('',*,*,#49449,.T.);
#65500=ORIENTED_EDGE('',*,*,#49450,.T.);
#65501=ORIENTED_EDGE('',*,*,#49451,.T.);
#65502=ORIENTED_EDGE('',*,*,#49452,.T.);
#65503=ORIENTED_EDGE('',*,*,#49453,.T.);
#65504=ORIENTED_EDGE('',*,*,#49454,.T.);
#65505=ORIENTED_EDGE('',*,*,#49455,.T.);
#65506=ORIENTED_EDGE('',*,*,#49456,.T.);
#65507=ORIENTED_EDGE('',*,*,#49457,.T.);
#65508=ORIENTED_EDGE('',*,*,#49458,.T.);
#65509=ORIENTED_EDGE('',*,*,#49459,.T.);
#65510=ORIENTED_EDGE('',*,*,#49460,.T.);
#65511=ORIENTED_EDGE('',*,*,#49461,.T.);
#65512=ORIENTED_EDGE('',*,*,#49462,.T.);
#65513=ORIENTED_EDGE('',*,*,#49463,.T.);
#65514=ORIENTED_EDGE('',*,*,#49464,.T.);
#65515=ORIENTED_EDGE('',*,*,#49465,.T.);
#65516=ORIENTED_EDGE('',*,*,#49466,.T.);
#65517=ORIENTED_EDGE('',*,*,#49467,.T.);
#65518=ORIENTED_EDGE('',*,*,#49468,.T.);
#65519=ORIENTED_EDGE('',*,*,#49469,.T.);
#65520=ORIENTED_EDGE('',*,*,#49470,.T.);
#65521=ORIENTED_EDGE('',*,*,#49471,.T.);
#65522=ORIENTED_EDGE('',*,*,#49472,.T.);
#65523=ORIENTED_EDGE('',*,*,#49473,.T.);
#65524=ORIENTED_EDGE('',*,*,#49474,.T.);
#65525=ORIENTED_EDGE('',*,*,#49475,.T.);
#65526=ORIENTED_EDGE('',*,*,#49476,.T.);
#65527=ORIENTED_EDGE('',*,*,#49477,.T.);
#65528=ORIENTED_EDGE('',*,*,#49478,.T.);
#65529=ORIENTED_EDGE('',*,*,#49479,.T.);
#65530=ORIENTED_EDGE('',*,*,#49480,.T.);
#65531=ORIENTED_EDGE('',*,*,#49481,.T.);
#65532=ORIENTED_EDGE('',*,*,#49482,.T.);
#65533=ORIENTED_EDGE('',*,*,#49483,.T.);
#65534=ORIENTED_EDGE('',*,*,#49484,.T.);
#65535=ORIENTED_EDGE('',*,*,#49485,.T.);
#65536=ORIENTED_EDGE('',*,*,#49486,.T.);
#65537=ORIENTED_EDGE('',*,*,#49487,.T.);
#65538=ORIENTED_EDGE('',*,*,#49488,.T.);
#65539=ORIENTED_EDGE('',*,*,#49489,.T.);
#65540=ORIENTED_EDGE('',*,*,#49490,.T.);
#65541=ORIENTED_EDGE('',*,*,#49491,.T.);
#65542=ORIENTED_EDGE('',*,*,#49492,.T.);
#65543=ORIENTED_EDGE('',*,*,#49493,.T.);
#65544=ORIENTED_EDGE('',*,*,#49494,.T.);
#65545=ORIENTED_EDGE('',*,*,#49495,.T.);
#65546=ORIENTED_EDGE('',*,*,#49496,.T.);
#65547=ORIENTED_EDGE('',*,*,#49497,.T.);
#65548=ORIENTED_EDGE('',*,*,#49498,.T.);
#65549=ORIENTED_EDGE('',*,*,#49499,.T.);
#65550=ORIENTED_EDGE('',*,*,#49500,.T.);
#65551=ORIENTED_EDGE('',*,*,#49501,.T.);
#65552=ORIENTED_EDGE('',*,*,#49502,.T.);
#65553=ORIENTED_EDGE('',*,*,#49503,.T.);
#65554=ORIENTED_EDGE('',*,*,#49504,.T.);
#65555=ORIENTED_EDGE('',*,*,#49505,.T.);
#65556=ORIENTED_EDGE('',*,*,#49506,.T.);
#65557=ORIENTED_EDGE('',*,*,#49507,.T.);
#65558=ORIENTED_EDGE('',*,*,#49508,.T.);
#65559=ORIENTED_EDGE('',*,*,#49509,.T.);
#65560=ORIENTED_EDGE('',*,*,#49510,.T.);
#65561=ORIENTED_EDGE('',*,*,#49511,.T.);
#65562=ORIENTED_EDGE('',*,*,#49512,.T.);
#65563=ORIENTED_EDGE('',*,*,#49513,.T.);
#65564=ORIENTED_EDGE('',*,*,#49514,.T.);
#65565=ORIENTED_EDGE('',*,*,#49515,.T.);
#65566=ORIENTED_EDGE('',*,*,#49516,.T.);
#65567=ORIENTED_EDGE('',*,*,#49517,.T.);
#65568=ORIENTED_EDGE('',*,*,#49518,.T.);
#65569=ORIENTED_EDGE('',*,*,#49519,.T.);
#65570=ORIENTED_EDGE('',*,*,#49520,.T.);
#65571=ORIENTED_EDGE('',*,*,#49521,.T.);
#65572=ORIENTED_EDGE('',*,*,#49522,.T.);
#65573=ORIENTED_EDGE('',*,*,#49523,.T.);
#65574=ORIENTED_EDGE('',*,*,#49524,.T.);
#65575=ORIENTED_EDGE('',*,*,#49525,.T.);
#65576=ORIENTED_EDGE('',*,*,#49526,.T.);
#65577=ORIENTED_EDGE('',*,*,#49527,.T.);
#65578=ORIENTED_EDGE('',*,*,#49528,.T.);
#65579=ORIENTED_EDGE('',*,*,#49529,.T.);
#65580=ORIENTED_EDGE('',*,*,#49530,.T.);
#65581=ORIENTED_EDGE('',*,*,#49531,.T.);
#65582=ORIENTED_EDGE('',*,*,#49532,.T.);
#65583=ORIENTED_EDGE('',*,*,#49533,.T.);
#65584=ORIENTED_EDGE('',*,*,#49534,.T.);
#65585=ORIENTED_EDGE('',*,*,#49535,.T.);
#65586=ORIENTED_EDGE('',*,*,#49536,.T.);
#65587=ORIENTED_EDGE('',*,*,#49537,.T.);
#65588=ORIENTED_EDGE('',*,*,#49538,.T.);
#65589=ORIENTED_EDGE('',*,*,#49539,.T.);
#65590=ORIENTED_EDGE('',*,*,#49540,.T.);
#65591=ORIENTED_EDGE('',*,*,#49541,.T.);
#65592=ORIENTED_EDGE('',*,*,#49542,.T.);
#65593=ORIENTED_EDGE('',*,*,#49543,.T.);
#65594=ORIENTED_EDGE('',*,*,#49544,.T.);
#65595=ORIENTED_EDGE('',*,*,#49545,.T.);
#65596=ORIENTED_EDGE('',*,*,#49546,.T.);
#65597=ORIENTED_EDGE('',*,*,#49547,.T.);
#65598=ORIENTED_EDGE('',*,*,#49548,.T.);
#65599=ORIENTED_EDGE('',*,*,#49549,.T.);
#65600=ORIENTED_EDGE('',*,*,#49550,.T.);
#65601=ORIENTED_EDGE('',*,*,#49551,.T.);
#65602=ORIENTED_EDGE('',*,*,#49552,.T.);
#65603=ORIENTED_EDGE('',*,*,#49553,.T.);
#65604=ORIENTED_EDGE('',*,*,#49554,.T.);
#65605=ORIENTED_EDGE('',*,*,#49555,.T.);
#65606=ORIENTED_EDGE('',*,*,#49556,.T.);
#65607=ORIENTED_EDGE('',*,*,#49557,.T.);
#65608=ORIENTED_EDGE('',*,*,#49558,.T.);
#65609=ORIENTED_EDGE('',*,*,#49559,.T.);
#65610=ORIENTED_EDGE('',*,*,#49560,.T.);
#65611=ORIENTED_EDGE('',*,*,#49561,.T.);
#65612=ORIENTED_EDGE('',*,*,#49562,.T.);
#65613=ORIENTED_EDGE('',*,*,#49563,.T.);
#65614=ORIENTED_EDGE('',*,*,#49564,.T.);
#65615=ORIENTED_EDGE('',*,*,#49565,.T.);
#65616=ORIENTED_EDGE('',*,*,#49566,.T.);
#65617=ORIENTED_EDGE('',*,*,#49567,.T.);
#65618=ORIENTED_EDGE('',*,*,#49568,.T.);
#65619=ORIENTED_EDGE('',*,*,#49569,.T.);
#65620=ORIENTED_EDGE('',*,*,#49570,.T.);
#65621=ORIENTED_EDGE('',*,*,#49571,.T.);
#65622=ORIENTED_EDGE('',*,*,#49572,.T.);
#65623=ORIENTED_EDGE('',*,*,#49573,.T.);
#65624=ORIENTED_EDGE('',*,*,#49574,.T.);
#65625=ORIENTED_EDGE('',*,*,#49575,.T.);
#65626=ORIENTED_EDGE('',*,*,#49576,.T.);
#65627=ORIENTED_EDGE('',*,*,#49577,.T.);
#65628=ORIENTED_EDGE('',*,*,#49578,.T.);
#65629=ORIENTED_EDGE('',*,*,#49579,.T.);
#65630=ORIENTED_EDGE('',*,*,#49580,.T.);
#65631=ORIENTED_EDGE('',*,*,#49581,.T.);
#65632=ORIENTED_EDGE('',*,*,#49582,.T.);
#65633=ORIENTED_EDGE('',*,*,#49583,.T.);
#65634=ORIENTED_EDGE('',*,*,#49584,.T.);
#65635=ORIENTED_EDGE('',*,*,#49585,.T.);
#65636=ORIENTED_EDGE('',*,*,#49586,.T.);
#65637=ORIENTED_EDGE('',*,*,#49587,.T.);
#65638=ORIENTED_EDGE('',*,*,#49588,.T.);
#65639=ORIENTED_EDGE('',*,*,#49589,.T.);
#65640=ORIENTED_EDGE('',*,*,#49590,.T.);
#65641=ORIENTED_EDGE('',*,*,#49591,.T.);
#65642=ORIENTED_EDGE('',*,*,#49592,.T.);
#65643=ORIENTED_EDGE('',*,*,#49593,.T.);
#65644=ORIENTED_EDGE('',*,*,#49594,.T.);
#65645=ORIENTED_EDGE('',*,*,#49595,.T.);
#65646=ORIENTED_EDGE('',*,*,#49596,.T.);
#65647=ORIENTED_EDGE('',*,*,#49597,.T.);
#65648=ORIENTED_EDGE('',*,*,#49598,.T.);
#65649=ORIENTED_EDGE('',*,*,#49599,.T.);
#65650=ORIENTED_EDGE('',*,*,#49600,.T.);
#65651=ORIENTED_EDGE('',*,*,#49601,.T.);
#65652=ORIENTED_EDGE('',*,*,#49602,.T.);
#65653=ORIENTED_EDGE('',*,*,#49603,.T.);
#65654=ORIENTED_EDGE('',*,*,#49604,.T.);
#65655=ORIENTED_EDGE('',*,*,#49605,.T.);
#65656=ORIENTED_EDGE('',*,*,#49606,.T.);
#65657=ORIENTED_EDGE('',*,*,#49607,.T.);
#65658=ORIENTED_EDGE('',*,*,#49608,.T.);
#65659=ORIENTED_EDGE('',*,*,#49609,.T.);
#65660=ORIENTED_EDGE('',*,*,#49610,.T.);
#65661=ORIENTED_EDGE('',*,*,#49611,.T.);
#65662=ORIENTED_EDGE('',*,*,#49612,.T.);
#65663=ORIENTED_EDGE('',*,*,#49613,.T.);
#65664=ORIENTED_EDGE('',*,*,#49614,.T.);
#65665=ORIENTED_EDGE('',*,*,#49615,.T.);
#65666=ORIENTED_EDGE('',*,*,#49616,.T.);
#65667=ORIENTED_EDGE('',*,*,#49617,.T.);
#65668=ORIENTED_EDGE('',*,*,#49618,.T.);
#65669=ORIENTED_EDGE('',*,*,#49619,.T.);
#65670=ORIENTED_EDGE('',*,*,#49620,.T.);
#65671=ORIENTED_EDGE('',*,*,#49621,.T.);
#65672=ORIENTED_EDGE('',*,*,#49622,.T.);
#65673=ORIENTED_EDGE('',*,*,#49623,.T.);
#65674=ORIENTED_EDGE('',*,*,#49624,.T.);
#65675=ORIENTED_EDGE('',*,*,#49625,.T.);
#65676=ORIENTED_EDGE('',*,*,#49626,.T.);
#65677=ORIENTED_EDGE('',*,*,#49627,.T.);
#65678=ORIENTED_EDGE('',*,*,#49628,.T.);
#65679=ORIENTED_EDGE('',*,*,#49629,.T.);
#65680=ORIENTED_EDGE('',*,*,#49630,.T.);
#65681=ORIENTED_EDGE('',*,*,#49631,.T.);
#65682=ORIENTED_EDGE('',*,*,#49632,.T.);
#65683=ORIENTED_EDGE('',*,*,#49633,.T.);
#65684=ORIENTED_EDGE('',*,*,#49634,.T.);
#65685=ORIENTED_EDGE('',*,*,#49635,.T.);
#65686=ORIENTED_EDGE('',*,*,#49636,.T.);
#65687=ORIENTED_EDGE('',*,*,#49637,.T.);
#65688=ORIENTED_EDGE('',*,*,#49638,.T.);
#65689=ORIENTED_EDGE('',*,*,#49639,.T.);
#65690=ORIENTED_EDGE('',*,*,#49640,.T.);
#65691=ORIENTED_EDGE('',*,*,#49641,.T.);
#65692=ORIENTED_EDGE('',*,*,#49642,.T.);
#65693=ORIENTED_EDGE('',*,*,#49643,.T.);
#65694=ORIENTED_EDGE('',*,*,#49644,.T.);
#65695=ORIENTED_EDGE('',*,*,#49645,.T.);
#65696=ORIENTED_EDGE('',*,*,#49646,.T.);
#65697=ORIENTED_EDGE('',*,*,#49647,.T.);
#65698=ORIENTED_EDGE('',*,*,#49648,.T.);
#65699=ORIENTED_EDGE('',*,*,#49649,.T.);
#65700=ORIENTED_EDGE('',*,*,#49650,.T.);
#65701=ORIENTED_EDGE('',*,*,#49651,.T.);
#65702=ORIENTED_EDGE('',*,*,#49652,.T.);
#65703=ORIENTED_EDGE('',*,*,#49653,.T.);
#65704=ORIENTED_EDGE('',*,*,#49654,.T.);
#65705=ORIENTED_EDGE('',*,*,#49655,.T.);
#65706=ORIENTED_EDGE('',*,*,#49656,.T.);
#65707=ORIENTED_EDGE('',*,*,#49657,.T.);
#65708=ORIENTED_EDGE('',*,*,#49658,.T.);
#65709=ORIENTED_EDGE('',*,*,#49659,.T.);
#65710=ORIENTED_EDGE('',*,*,#49660,.T.);
#65711=ORIENTED_EDGE('',*,*,#49661,.T.);
#65712=ORIENTED_EDGE('',*,*,#49662,.T.);
#65713=ORIENTED_EDGE('',*,*,#49663,.T.);
#65714=ORIENTED_EDGE('',*,*,#49664,.T.);
#65715=ORIENTED_EDGE('',*,*,#49665,.T.);
#65716=ORIENTED_EDGE('',*,*,#49666,.T.);
#65717=ORIENTED_EDGE('',*,*,#49667,.T.);
#65718=ORIENTED_EDGE('',*,*,#49668,.T.);
#65719=ORIENTED_EDGE('',*,*,#49669,.T.);
#65720=ORIENTED_EDGE('',*,*,#49670,.T.);
#65721=ORIENTED_EDGE('',*,*,#49671,.T.);
#65722=ORIENTED_EDGE('',*,*,#49672,.T.);
#65723=ORIENTED_EDGE('',*,*,#49673,.T.);
#65724=ORIENTED_EDGE('',*,*,#49674,.T.);
#65725=ORIENTED_EDGE('',*,*,#49675,.T.);
#65726=ORIENTED_EDGE('',*,*,#49676,.T.);
#65727=ORIENTED_EDGE('',*,*,#49677,.T.);
#65728=ORIENTED_EDGE('',*,*,#49678,.T.);
#65729=ORIENTED_EDGE('',*,*,#49679,.T.);
#65730=ORIENTED_EDGE('',*,*,#49680,.T.);
#65731=ORIENTED_EDGE('',*,*,#49681,.T.);
#65732=ORIENTED_EDGE('',*,*,#49682,.T.);
#65733=ORIENTED_EDGE('',*,*,#49683,.T.);
#65734=ORIENTED_EDGE('',*,*,#49684,.T.);
#65735=ORIENTED_EDGE('',*,*,#49685,.T.);
#65736=ORIENTED_EDGE('',*,*,#49686,.T.);
#65737=ORIENTED_EDGE('',*,*,#49687,.T.);
#65738=ORIENTED_EDGE('',*,*,#49688,.T.);
#65739=ORIENTED_EDGE('',*,*,#49689,.T.);
#65740=ORIENTED_EDGE('',*,*,#49690,.T.);
#65741=ORIENTED_EDGE('',*,*,#49691,.T.);
#65742=ORIENTED_EDGE('',*,*,#49692,.T.);
#65743=ORIENTED_EDGE('',*,*,#49693,.T.);
#65744=ORIENTED_EDGE('',*,*,#49694,.T.);
#65745=ORIENTED_EDGE('',*,*,#49695,.T.);
#65746=ORIENTED_EDGE('',*,*,#49696,.T.);
#65747=ORIENTED_EDGE('',*,*,#49697,.T.);
#65748=ORIENTED_EDGE('',*,*,#49698,.T.);
#65749=ORIENTED_EDGE('',*,*,#49699,.T.);
#65750=ORIENTED_EDGE('',*,*,#49700,.T.);
#65751=ORIENTED_EDGE('',*,*,#49701,.T.);
#65752=ORIENTED_EDGE('',*,*,#49702,.T.);
#65753=ORIENTED_EDGE('',*,*,#49703,.T.);
#65754=ORIENTED_EDGE('',*,*,#49704,.T.);
#65755=ORIENTED_EDGE('',*,*,#49705,.T.);
#65756=ORIENTED_EDGE('',*,*,#49706,.T.);
#65757=ORIENTED_EDGE('',*,*,#49707,.T.);
#65758=ORIENTED_EDGE('',*,*,#49708,.T.);
#65759=ORIENTED_EDGE('',*,*,#49709,.T.);
#65760=ORIENTED_EDGE('',*,*,#49710,.T.);
#65761=ORIENTED_EDGE('',*,*,#49711,.T.);
#65762=ORIENTED_EDGE('',*,*,#49712,.T.);
#65763=ORIENTED_EDGE('',*,*,#49713,.T.);
#65764=ORIENTED_EDGE('',*,*,#49714,.T.);
#65765=ORIENTED_EDGE('',*,*,#49715,.T.);
#65766=ORIENTED_EDGE('',*,*,#49716,.T.);
#65767=ORIENTED_EDGE('',*,*,#49717,.T.);
#65768=ORIENTED_EDGE('',*,*,#49718,.T.);
#65769=ORIENTED_EDGE('',*,*,#49719,.T.);
#65770=ORIENTED_EDGE('',*,*,#49720,.T.);
#65771=ORIENTED_EDGE('',*,*,#49721,.T.);
#65772=ORIENTED_EDGE('',*,*,#49722,.T.);
#65773=ORIENTED_EDGE('',*,*,#49723,.T.);
#65774=ORIENTED_EDGE('',*,*,#49724,.T.);
#65775=ORIENTED_EDGE('',*,*,#49725,.T.);
#65776=ORIENTED_EDGE('',*,*,#49726,.T.);
#65777=ORIENTED_EDGE('',*,*,#49727,.T.);
#65778=ORIENTED_EDGE('',*,*,#49728,.T.);
#65779=ORIENTED_EDGE('',*,*,#49729,.T.);
#65780=ORIENTED_EDGE('',*,*,#49730,.T.);
#65781=ORIENTED_EDGE('',*,*,#49731,.T.);
#65782=ORIENTED_EDGE('',*,*,#45888,.T.);
#65783=ORIENTED_EDGE('',*,*,#49732,.T.);
#65784=ORIENTED_EDGE('',*,*,#45882,.T.);
#65785=ORIENTED_EDGE('',*,*,#49733,.T.);
#65786=ORIENTED_EDGE('',*,*,#49734,.T.);
#65787=ORIENTED_EDGE('',*,*,#49735,.T.);
#65788=ORIENTED_EDGE('',*,*,#49736,.T.);
#65789=ORIENTED_EDGE('',*,*,#49737,.T.);
#65790=ORIENTED_EDGE('',*,*,#49738,.T.);
#65791=ORIENTED_EDGE('',*,*,#49739,.T.);
#65792=ORIENTED_EDGE('',*,*,#49740,.T.);
#65793=ORIENTED_EDGE('',*,*,#49741,.T.);
#65794=ORIENTED_EDGE('',*,*,#49742,.T.);
#65795=ORIENTED_EDGE('',*,*,#49743,.T.);
#65796=ORIENTED_EDGE('',*,*,#49744,.T.);
#65797=ORIENTED_EDGE('',*,*,#49745,.T.);
#65798=ORIENTED_EDGE('',*,*,#49746,.T.);
#65799=ORIENTED_EDGE('',*,*,#49747,.T.);
#65800=ORIENTED_EDGE('',*,*,#49748,.T.);
#65801=ORIENTED_EDGE('',*,*,#49749,.T.);
#65802=ORIENTED_EDGE('',*,*,#49750,.T.);
#65803=ORIENTED_EDGE('',*,*,#49751,.T.);
#65804=ORIENTED_EDGE('',*,*,#49752,.T.);
#65805=ORIENTED_EDGE('',*,*,#49753,.T.);
#65806=ORIENTED_EDGE('',*,*,#49754,.T.);
#65807=ORIENTED_EDGE('',*,*,#49755,.T.);
#65808=ORIENTED_EDGE('',*,*,#49756,.T.);
#65809=ORIENTED_EDGE('',*,*,#49757,.T.);
#65810=ORIENTED_EDGE('',*,*,#49758,.T.);
#65811=ORIENTED_EDGE('',*,*,#49759,.T.);
#65812=ORIENTED_EDGE('',*,*,#49760,.T.);
#65813=ORIENTED_EDGE('',*,*,#49761,.T.);
#65814=ORIENTED_EDGE('',*,*,#49762,.T.);
#65815=ORIENTED_EDGE('',*,*,#49763,.T.);
#65816=ORIENTED_EDGE('',*,*,#49764,.T.);
#65817=ORIENTED_EDGE('',*,*,#49765,.T.);
#65818=ORIENTED_EDGE('',*,*,#49766,.T.);
#65819=ORIENTED_EDGE('',*,*,#49767,.T.);
#65820=ORIENTED_EDGE('',*,*,#49768,.T.);
#65821=ORIENTED_EDGE('',*,*,#49769,.T.);
#65822=ORIENTED_EDGE('',*,*,#49770,.T.);
#65823=ORIENTED_EDGE('',*,*,#49771,.T.);
#65824=ORIENTED_EDGE('',*,*,#49772,.T.);
#65825=ORIENTED_EDGE('',*,*,#49773,.T.);
#65826=ORIENTED_EDGE('',*,*,#49774,.T.);
#65827=ORIENTED_EDGE('',*,*,#49775,.T.);
#65828=ORIENTED_EDGE('',*,*,#49776,.T.);
#65829=ORIENTED_EDGE('',*,*,#49777,.T.);
#65830=ORIENTED_EDGE('',*,*,#49778,.T.);
#65831=ORIENTED_EDGE('',*,*,#49779,.T.);
#65832=ORIENTED_EDGE('',*,*,#49780,.T.);
#65833=ORIENTED_EDGE('',*,*,#49781,.T.);
#65834=ORIENTED_EDGE('',*,*,#49782,.T.);
#65835=ORIENTED_EDGE('',*,*,#49783,.T.);
#65836=ORIENTED_EDGE('',*,*,#49784,.T.);
#65837=ORIENTED_EDGE('',*,*,#49785,.T.);
#65838=ORIENTED_EDGE('',*,*,#49786,.T.);
#65839=ORIENTED_EDGE('',*,*,#49787,.T.);
#65840=ORIENTED_EDGE('',*,*,#49788,.T.);
#65841=ORIENTED_EDGE('',*,*,#49789,.T.);
#65842=ORIENTED_EDGE('',*,*,#49790,.T.);
#65843=ORIENTED_EDGE('',*,*,#49791,.T.);
#65844=ORIENTED_EDGE('',*,*,#49792,.T.);
#65845=ORIENTED_EDGE('',*,*,#49793,.T.);
#65846=ORIENTED_EDGE('',*,*,#49794,.T.);
#65847=ORIENTED_EDGE('',*,*,#49795,.T.);
#65848=ORIENTED_EDGE('',*,*,#49796,.T.);
#65849=ORIENTED_EDGE('',*,*,#49797,.T.);
#65850=ORIENTED_EDGE('',*,*,#49798,.T.);
#65851=ORIENTED_EDGE('',*,*,#49799,.T.);
#65852=ORIENTED_EDGE('',*,*,#49800,.T.);
#65853=ORIENTED_EDGE('',*,*,#49801,.T.);
#65854=ORIENTED_EDGE('',*,*,#49802,.T.);
#65855=ORIENTED_EDGE('',*,*,#49803,.T.);
#65856=ORIENTED_EDGE('',*,*,#49804,.T.);
#65857=ORIENTED_EDGE('',*,*,#49805,.T.);
#65858=ORIENTED_EDGE('',*,*,#49806,.T.);
#65859=ORIENTED_EDGE('',*,*,#49807,.T.);
#65860=ORIENTED_EDGE('',*,*,#49808,.T.);
#65861=ORIENTED_EDGE('',*,*,#49809,.T.);
#65862=ORIENTED_EDGE('',*,*,#49810,.T.);
#65863=ORIENTED_EDGE('',*,*,#49811,.T.);
#65864=ORIENTED_EDGE('',*,*,#49812,.T.);
#65865=ORIENTED_EDGE('',*,*,#49813,.T.);
#65866=ORIENTED_EDGE('',*,*,#49814,.T.);
#65867=ORIENTED_EDGE('',*,*,#49815,.T.);
#65868=ORIENTED_EDGE('',*,*,#49816,.T.);
#65869=ORIENTED_EDGE('',*,*,#49817,.T.);
#65870=ORIENTED_EDGE('',*,*,#49818,.T.);
#65871=ORIENTED_EDGE('',*,*,#49819,.T.);
#65872=ORIENTED_EDGE('',*,*,#49820,.T.);
#65873=ORIENTED_EDGE('',*,*,#49821,.T.);
#65874=ORIENTED_EDGE('',*,*,#49822,.T.);
#65875=ORIENTED_EDGE('',*,*,#49823,.T.);
#65876=ORIENTED_EDGE('',*,*,#49824,.T.);
#65877=ORIENTED_EDGE('',*,*,#49825,.T.);
#65878=ORIENTED_EDGE('',*,*,#49826,.T.);
#65879=ORIENTED_EDGE('',*,*,#49827,.T.);
#65880=ORIENTED_EDGE('',*,*,#49828,.T.);
#65881=ORIENTED_EDGE('',*,*,#49829,.T.);
#65882=ORIENTED_EDGE('',*,*,#49830,.T.);
#65883=ORIENTED_EDGE('',*,*,#49831,.T.);
#65884=ORIENTED_EDGE('',*,*,#49832,.T.);
#65885=ORIENTED_EDGE('',*,*,#49833,.T.);
#65886=ORIENTED_EDGE('',*,*,#49834,.T.);
#65887=ORIENTED_EDGE('',*,*,#49835,.T.);
#65888=ORIENTED_EDGE('',*,*,#49836,.T.);
#65889=ORIENTED_EDGE('',*,*,#49837,.T.);
#65890=ORIENTED_EDGE('',*,*,#49838,.T.);
#65891=ORIENTED_EDGE('',*,*,#49839,.T.);
#65892=ORIENTED_EDGE('',*,*,#49840,.T.);
#65893=ORIENTED_EDGE('',*,*,#49841,.T.);
#65894=ORIENTED_EDGE('',*,*,#49842,.T.);
#65895=ORIENTED_EDGE('',*,*,#49843,.T.);
#65896=ORIENTED_EDGE('',*,*,#49844,.T.);
#65897=ORIENTED_EDGE('',*,*,#49845,.T.);
#65898=ORIENTED_EDGE('',*,*,#49846,.T.);
#65899=ORIENTED_EDGE('',*,*,#49847,.T.);
#65900=ORIENTED_EDGE('',*,*,#49848,.T.);
#65901=ORIENTED_EDGE('',*,*,#49849,.T.);
#65902=ORIENTED_EDGE('',*,*,#49850,.T.);
#65903=ORIENTED_EDGE('',*,*,#49851,.T.);
#65904=ORIENTED_EDGE('',*,*,#49852,.T.);
#65905=ORIENTED_EDGE('',*,*,#49853,.T.);
#65906=ORIENTED_EDGE('',*,*,#49854,.T.);
#65907=ORIENTED_EDGE('',*,*,#49855,.T.);
#65908=ORIENTED_EDGE('',*,*,#49856,.T.);
#65909=ORIENTED_EDGE('',*,*,#49857,.T.);
#65910=ORIENTED_EDGE('',*,*,#49858,.T.);
#65911=ORIENTED_EDGE('',*,*,#49859,.T.);
#65912=ORIENTED_EDGE('',*,*,#49860,.T.);
#65913=ORIENTED_EDGE('',*,*,#49861,.T.);
#65914=ORIENTED_EDGE('',*,*,#49862,.T.);
#65915=ORIENTED_EDGE('',*,*,#49863,.T.);
#65916=ORIENTED_EDGE('',*,*,#49864,.T.);
#65917=ORIENTED_EDGE('',*,*,#49865,.T.);
#65918=ORIENTED_EDGE('',*,*,#49866,.T.);
#65919=ORIENTED_EDGE('',*,*,#49867,.T.);
#65920=ORIENTED_EDGE('',*,*,#49868,.T.);
#65921=ORIENTED_EDGE('',*,*,#49869,.T.);
#65922=ORIENTED_EDGE('',*,*,#49870,.T.);
#65923=ORIENTED_EDGE('',*,*,#49871,.T.);
#65924=ORIENTED_EDGE('',*,*,#49872,.T.);
#65925=ORIENTED_EDGE('',*,*,#49873,.T.);
#65926=ORIENTED_EDGE('',*,*,#49874,.T.);
#65927=ORIENTED_EDGE('',*,*,#49875,.T.);
#65928=ORIENTED_EDGE('',*,*,#49876,.T.);
#65929=ORIENTED_EDGE('',*,*,#49877,.T.);
#65930=ORIENTED_EDGE('',*,*,#49878,.T.);
#65931=ORIENTED_EDGE('',*,*,#49879,.T.);
#65932=ORIENTED_EDGE('',*,*,#49880,.T.);
#65933=ORIENTED_EDGE('',*,*,#49881,.T.);
#65934=ORIENTED_EDGE('',*,*,#49882,.T.);
#65935=ORIENTED_EDGE('',*,*,#49883,.T.);
#65936=ORIENTED_EDGE('',*,*,#49884,.T.);
#65937=ORIENTED_EDGE('',*,*,#49885,.T.);
#65938=ORIENTED_EDGE('',*,*,#49886,.T.);
#65939=ORIENTED_EDGE('',*,*,#49887,.T.);
#65940=ORIENTED_EDGE('',*,*,#49888,.T.);
#65941=ORIENTED_EDGE('',*,*,#49889,.T.);
#65942=ORIENTED_EDGE('',*,*,#49890,.T.);
#65943=ORIENTED_EDGE('',*,*,#49891,.T.);
#65944=ORIENTED_EDGE('',*,*,#49892,.T.);
#65945=ORIENTED_EDGE('',*,*,#49893,.T.);
#65946=ORIENTED_EDGE('',*,*,#49894,.T.);
#65947=ORIENTED_EDGE('',*,*,#49895,.T.);
#65948=ORIENTED_EDGE('',*,*,#49896,.T.);
#65949=ORIENTED_EDGE('',*,*,#49897,.T.);
#65950=ORIENTED_EDGE('',*,*,#49898,.T.);
#65951=ORIENTED_EDGE('',*,*,#49899,.T.);
#65952=ORIENTED_EDGE('',*,*,#49900,.T.);
#65953=ORIENTED_EDGE('',*,*,#49901,.T.);
#65954=ORIENTED_EDGE('',*,*,#49902,.T.);
#65955=ORIENTED_EDGE('',*,*,#49903,.T.);
#65956=ORIENTED_EDGE('',*,*,#49904,.T.);
#65957=ORIENTED_EDGE('',*,*,#49905,.T.);
#65958=ORIENTED_EDGE('',*,*,#49906,.T.);
#65959=ORIENTED_EDGE('',*,*,#49907,.T.);
#65960=ORIENTED_EDGE('',*,*,#49908,.T.);
#65961=ORIENTED_EDGE('',*,*,#49909,.T.);
#65962=ORIENTED_EDGE('',*,*,#49910,.T.);
#65963=ORIENTED_EDGE('',*,*,#49911,.T.);
#65964=ORIENTED_EDGE('',*,*,#49912,.T.);
#65965=ORIENTED_EDGE('',*,*,#49913,.T.);
#65966=ORIENTED_EDGE('',*,*,#49914,.T.);
#65967=ORIENTED_EDGE('',*,*,#49915,.T.);
#65968=ORIENTED_EDGE('',*,*,#49916,.T.);
#65969=ORIENTED_EDGE('',*,*,#49917,.T.);
#65970=ORIENTED_EDGE('',*,*,#49918,.T.);
#65971=ORIENTED_EDGE('',*,*,#49919,.T.);
#65972=ORIENTED_EDGE('',*,*,#49920,.T.);
#65973=ORIENTED_EDGE('',*,*,#49921,.T.);
#65974=ORIENTED_EDGE('',*,*,#49922,.T.);
#65975=ORIENTED_EDGE('',*,*,#49923,.T.);
#65976=ORIENTED_EDGE('',*,*,#49924,.T.);
#65977=ORIENTED_EDGE('',*,*,#49925,.T.);
#65978=ORIENTED_EDGE('',*,*,#49926,.T.);
#65979=ORIENTED_EDGE('',*,*,#49927,.T.);
#65980=ORIENTED_EDGE('',*,*,#49928,.T.);
#65981=ORIENTED_EDGE('',*,*,#49929,.T.);
#65982=ORIENTED_EDGE('',*,*,#49930,.T.);
#65983=ORIENTED_EDGE('',*,*,#49931,.T.);
#65984=ORIENTED_EDGE('',*,*,#49932,.T.);
#65985=ORIENTED_EDGE('',*,*,#49933,.T.);
#65986=ORIENTED_EDGE('',*,*,#49934,.T.);
#65987=ORIENTED_EDGE('',*,*,#49935,.T.);
#65988=ORIENTED_EDGE('',*,*,#49936,.T.);
#65989=ORIENTED_EDGE('',*,*,#49937,.T.);
#65990=ORIENTED_EDGE('',*,*,#49938,.T.);
#65991=ORIENTED_EDGE('',*,*,#49939,.T.);
#65992=ORIENTED_EDGE('',*,*,#49940,.T.);
#65993=ORIENTED_EDGE('',*,*,#49941,.T.);
#65994=ORIENTED_EDGE('',*,*,#49942,.T.);
#65995=ORIENTED_EDGE('',*,*,#49943,.T.);
#65996=ORIENTED_EDGE('',*,*,#49944,.T.);
#65997=ORIENTED_EDGE('',*,*,#49945,.T.);
#65998=ORIENTED_EDGE('',*,*,#49946,.T.);
#65999=ORIENTED_EDGE('',*,*,#49947,.T.);
#66000=ORIENTED_EDGE('',*,*,#49948,.T.);
#66001=ORIENTED_EDGE('',*,*,#49949,.T.);
#66002=ORIENTED_EDGE('',*,*,#49950,.T.);
#66003=ORIENTED_EDGE('',*,*,#49951,.T.);
#66004=ORIENTED_EDGE('',*,*,#49952,.T.);
#66005=ORIENTED_EDGE('',*,*,#49953,.T.);
#66006=ORIENTED_EDGE('',*,*,#49954,.T.);
#66007=ORIENTED_EDGE('',*,*,#49955,.T.);
#66008=ORIENTED_EDGE('',*,*,#49956,.T.);
#66009=ORIENTED_EDGE('',*,*,#49957,.T.);
#66010=ORIENTED_EDGE('',*,*,#49958,.T.);
#66011=ORIENTED_EDGE('',*,*,#49959,.T.);
#66012=ORIENTED_EDGE('',*,*,#49960,.T.);
#66013=ORIENTED_EDGE('',*,*,#49961,.T.);
#66014=ORIENTED_EDGE('',*,*,#49962,.T.);
#66015=ORIENTED_EDGE('',*,*,#49963,.T.);
#66016=ORIENTED_EDGE('',*,*,#49964,.T.);
#66017=ORIENTED_EDGE('',*,*,#49965,.T.);
#66018=ORIENTED_EDGE('',*,*,#49966,.T.);
#66019=ORIENTED_EDGE('',*,*,#49967,.T.);
#66020=ORIENTED_EDGE('',*,*,#49968,.T.);
#66021=ORIENTED_EDGE('',*,*,#49969,.T.);
#66022=ORIENTED_EDGE('',*,*,#49970,.T.);
#66023=ORIENTED_EDGE('',*,*,#49971,.T.);
#66024=ORIENTED_EDGE('',*,*,#49972,.T.);
#66025=ORIENTED_EDGE('',*,*,#49973,.T.);
#66026=ORIENTED_EDGE('',*,*,#49974,.T.);
#66027=ORIENTED_EDGE('',*,*,#49975,.T.);
#66028=ORIENTED_EDGE('',*,*,#49976,.T.);
#66029=ORIENTED_EDGE('',*,*,#49977,.T.);
#66030=ORIENTED_EDGE('',*,*,#49978,.T.);
#66031=ORIENTED_EDGE('',*,*,#49979,.T.);
#66032=ORIENTED_EDGE('',*,*,#49980,.T.);
#66033=ORIENTED_EDGE('',*,*,#49981,.T.);
#66034=ORIENTED_EDGE('',*,*,#49982,.T.);
#66035=ORIENTED_EDGE('',*,*,#49983,.T.);
#66036=ORIENTED_EDGE('',*,*,#49984,.T.);
#66037=ORIENTED_EDGE('',*,*,#49985,.T.);
#66038=ORIENTED_EDGE('',*,*,#49986,.T.);
#66039=ORIENTED_EDGE('',*,*,#49987,.T.);
#66040=ORIENTED_EDGE('',*,*,#49988,.T.);
#66041=ORIENTED_EDGE('',*,*,#49989,.T.);
#66042=ORIENTED_EDGE('',*,*,#49990,.T.);
#66043=ORIENTED_EDGE('',*,*,#49991,.T.);
#66044=ORIENTED_EDGE('',*,*,#49992,.T.);
#66045=ORIENTED_EDGE('',*,*,#49993,.T.);
#66046=ORIENTED_EDGE('',*,*,#49994,.T.);
#66047=ORIENTED_EDGE('',*,*,#49995,.T.);
#66048=ORIENTED_EDGE('',*,*,#49996,.T.);
#66049=ORIENTED_EDGE('',*,*,#49997,.T.);
#66050=ORIENTED_EDGE('',*,*,#49998,.T.);
#66051=ORIENTED_EDGE('',*,*,#49999,.T.);
#66052=ORIENTED_EDGE('',*,*,#50000,.T.);
#66053=ORIENTED_EDGE('',*,*,#50001,.T.);
#66054=ORIENTED_EDGE('',*,*,#50002,.T.);
#66055=ORIENTED_EDGE('',*,*,#50003,.T.);
#66056=ORIENTED_EDGE('',*,*,#50004,.T.);
#66057=ORIENTED_EDGE('',*,*,#50005,.T.);
#66058=ORIENTED_EDGE('',*,*,#50006,.T.);
#66059=ORIENTED_EDGE('',*,*,#50007,.T.);
#66060=ORIENTED_EDGE('',*,*,#50008,.T.);
#66061=ORIENTED_EDGE('',*,*,#50009,.T.);
#66062=ORIENTED_EDGE('',*,*,#50010,.T.);
#66063=ORIENTED_EDGE('',*,*,#50011,.T.);
#66064=ORIENTED_EDGE('',*,*,#50012,.T.);
#66065=ORIENTED_EDGE('',*,*,#50013,.T.);
#66066=ORIENTED_EDGE('',*,*,#50014,.T.);
#66067=ORIENTED_EDGE('',*,*,#50015,.T.);
#66068=ORIENTED_EDGE('',*,*,#50016,.T.);
#66069=ORIENTED_EDGE('',*,*,#50017,.T.);
#66070=ORIENTED_EDGE('',*,*,#50018,.T.);
#66071=ORIENTED_EDGE('',*,*,#50019,.T.);
#66072=ORIENTED_EDGE('',*,*,#50020,.T.);
#66073=ORIENTED_EDGE('',*,*,#50021,.T.);
#66074=ORIENTED_EDGE('',*,*,#50022,.T.);
#66075=ORIENTED_EDGE('',*,*,#50023,.T.);
#66076=ORIENTED_EDGE('',*,*,#50024,.T.);
#66077=ORIENTED_EDGE('',*,*,#50025,.T.);
#66078=ORIENTED_EDGE('',*,*,#50026,.T.);
#66079=ORIENTED_EDGE('',*,*,#50027,.T.);
#66080=ORIENTED_EDGE('',*,*,#50028,.T.);
#66081=ORIENTED_EDGE('',*,*,#50029,.T.);
#66082=ORIENTED_EDGE('',*,*,#50030,.T.);
#66083=ORIENTED_EDGE('',*,*,#50031,.T.);
#66084=ORIENTED_EDGE('',*,*,#50032,.T.);
#66085=ORIENTED_EDGE('',*,*,#50033,.T.);
#66086=ORIENTED_EDGE('',*,*,#50034,.T.);
#66087=ORIENTED_EDGE('',*,*,#50035,.T.);
#66088=ORIENTED_EDGE('',*,*,#50036,.T.);
#66089=ORIENTED_EDGE('',*,*,#50037,.T.);
#66090=ORIENTED_EDGE('',*,*,#50038,.T.);
#66091=ORIENTED_EDGE('',*,*,#50039,.T.);
#66092=ORIENTED_EDGE('',*,*,#50040,.T.);
#66093=ORIENTED_EDGE('',*,*,#50041,.T.);
#66094=ORIENTED_EDGE('',*,*,#50042,.T.);
#66095=ORIENTED_EDGE('',*,*,#50043,.T.);
#66096=ORIENTED_EDGE('',*,*,#50044,.T.);
#66097=ORIENTED_EDGE('',*,*,#50045,.T.);
#66098=ORIENTED_EDGE('',*,*,#50046,.T.);
#66099=ORIENTED_EDGE('',*,*,#50047,.T.);
#66100=ORIENTED_EDGE('',*,*,#50048,.T.);
#66101=ORIENTED_EDGE('',*,*,#50049,.T.);
#66102=ORIENTED_EDGE('',*,*,#50050,.T.);
#66103=ORIENTED_EDGE('',*,*,#50051,.T.);
#66104=ORIENTED_EDGE('',*,*,#50052,.T.);
#66105=ORIENTED_EDGE('',*,*,#50053,.T.);
#66106=ORIENTED_EDGE('',*,*,#50054,.T.);
#66107=ORIENTED_EDGE('',*,*,#50055,.T.);
#66108=ORIENTED_EDGE('',*,*,#50056,.T.);
#66109=ORIENTED_EDGE('',*,*,#50057,.T.);
#66110=ORIENTED_EDGE('',*,*,#50058,.T.);
#66111=ORIENTED_EDGE('',*,*,#50059,.T.);
#66112=ORIENTED_EDGE('',*,*,#50060,.T.);
#66113=ORIENTED_EDGE('',*,*,#50061,.T.);
#66114=ORIENTED_EDGE('',*,*,#50062,.T.);
#66115=ORIENTED_EDGE('',*,*,#50063,.T.);
#66116=ORIENTED_EDGE('',*,*,#50064,.T.);
#66117=ORIENTED_EDGE('',*,*,#50065,.T.);
#66118=ORIENTED_EDGE('',*,*,#50066,.T.);
#66119=ORIENTED_EDGE('',*,*,#50067,.T.);
#66120=ORIENTED_EDGE('',*,*,#50068,.T.);
#66121=ORIENTED_EDGE('',*,*,#50069,.T.);
#66122=ORIENTED_EDGE('',*,*,#50070,.T.);
#66123=ORIENTED_EDGE('',*,*,#50071,.T.);
#66124=ORIENTED_EDGE('',*,*,#50072,.T.);
#66125=ORIENTED_EDGE('',*,*,#50073,.T.);
#66126=ORIENTED_EDGE('',*,*,#50074,.T.);
#66127=ORIENTED_EDGE('',*,*,#50075,.T.);
#66128=ORIENTED_EDGE('',*,*,#50076,.T.);
#66129=ORIENTED_EDGE('',*,*,#50077,.T.);
#66130=ORIENTED_EDGE('',*,*,#50078,.T.);
#66131=ORIENTED_EDGE('',*,*,#50079,.T.);
#66132=ORIENTED_EDGE('',*,*,#50080,.T.);
#66133=ORIENTED_EDGE('',*,*,#50081,.T.);
#66134=ORIENTED_EDGE('',*,*,#50082,.T.);
#66135=ORIENTED_EDGE('',*,*,#50083,.T.);
#66136=ORIENTED_EDGE('',*,*,#50084,.T.);
#66137=ORIENTED_EDGE('',*,*,#50085,.T.);
#66138=ORIENTED_EDGE('',*,*,#50086,.T.);
#66139=ORIENTED_EDGE('',*,*,#50087,.T.);
#66140=ORIENTED_EDGE('',*,*,#50088,.T.);
#66141=ORIENTED_EDGE('',*,*,#50089,.T.);
#66142=ORIENTED_EDGE('',*,*,#50090,.T.);
#66143=ORIENTED_EDGE('',*,*,#50091,.T.);
#66144=ORIENTED_EDGE('',*,*,#50092,.T.);
#66145=ORIENTED_EDGE('',*,*,#50093,.T.);
#66146=ORIENTED_EDGE('',*,*,#50094,.T.);
#66147=ORIENTED_EDGE('',*,*,#50095,.T.);
#66148=ORIENTED_EDGE('',*,*,#50096,.T.);
#66149=ORIENTED_EDGE('',*,*,#50097,.T.);
#66150=ORIENTED_EDGE('',*,*,#50098,.T.);
#66151=ORIENTED_EDGE('',*,*,#50099,.T.);
#66152=ORIENTED_EDGE('',*,*,#50100,.T.);
#66153=ORIENTED_EDGE('',*,*,#50101,.T.);
#66154=ORIENTED_EDGE('',*,*,#50102,.T.);
#66155=ORIENTED_EDGE('',*,*,#50103,.T.);
#66156=ORIENTED_EDGE('',*,*,#50104,.T.);
#66157=ORIENTED_EDGE('',*,*,#50105,.T.);
#66158=ORIENTED_EDGE('',*,*,#50106,.T.);
#66159=ORIENTED_EDGE('',*,*,#50107,.T.);
#66160=ORIENTED_EDGE('',*,*,#50108,.T.);
#66161=ORIENTED_EDGE('',*,*,#50109,.T.);
#66162=ORIENTED_EDGE('',*,*,#50110,.T.);
#66163=ORIENTED_EDGE('',*,*,#50111,.T.);
#66164=ORIENTED_EDGE('',*,*,#50112,.T.);
#66165=ORIENTED_EDGE('',*,*,#50113,.T.);
#66166=ORIENTED_EDGE('',*,*,#50114,.T.);
#66167=ORIENTED_EDGE('',*,*,#50115,.T.);
#66168=ORIENTED_EDGE('',*,*,#50116,.T.);
#66169=ORIENTED_EDGE('',*,*,#50117,.T.);
#66170=ORIENTED_EDGE('',*,*,#50118,.T.);
#66171=ORIENTED_EDGE('',*,*,#50119,.T.);
#66172=ORIENTED_EDGE('',*,*,#50120,.T.);
#66173=ORIENTED_EDGE('',*,*,#50121,.T.);
#66174=ORIENTED_EDGE('',*,*,#50122,.T.);
#66175=ORIENTED_EDGE('',*,*,#50123,.T.);
#66176=ORIENTED_EDGE('',*,*,#50124,.T.);
#66177=ORIENTED_EDGE('',*,*,#50125,.T.);
#66178=ORIENTED_EDGE('',*,*,#50126,.T.);
#66179=ORIENTED_EDGE('',*,*,#50127,.T.);
#66180=ORIENTED_EDGE('',*,*,#50128,.T.);
#66181=ORIENTED_EDGE('',*,*,#50129,.T.);
#66182=ORIENTED_EDGE('',*,*,#50130,.T.);
#66183=ORIENTED_EDGE('',*,*,#50131,.T.);
#66184=ORIENTED_EDGE('',*,*,#50132,.T.);
#66185=ORIENTED_EDGE('',*,*,#50133,.T.);
#66186=ORIENTED_EDGE('',*,*,#50134,.T.);
#66187=ORIENTED_EDGE('',*,*,#50135,.T.);
#66188=ORIENTED_EDGE('',*,*,#50136,.T.);
#66189=ORIENTED_EDGE('',*,*,#50137,.T.);
#66190=ORIENTED_EDGE('',*,*,#50138,.T.);
#66191=ORIENTED_EDGE('',*,*,#50139,.T.);
#66192=ORIENTED_EDGE('',*,*,#50140,.T.);
#66193=ORIENTED_EDGE('',*,*,#50141,.T.);
#66194=ORIENTED_EDGE('',*,*,#50142,.T.);
#66195=ORIENTED_EDGE('',*,*,#50143,.T.);
#66196=ORIENTED_EDGE('',*,*,#50144,.T.);
#66197=ORIENTED_EDGE('',*,*,#50145,.T.);
#66198=ORIENTED_EDGE('',*,*,#50146,.T.);
#66199=ORIENTED_EDGE('',*,*,#50147,.T.);
#66200=ORIENTED_EDGE('',*,*,#50148,.T.);
#66201=ORIENTED_EDGE('',*,*,#48519,.F.);
#66202=ORIENTED_EDGE('',*,*,#50149,.T.);
#66203=ORIENTED_EDGE('',*,*,#48501,.F.);
#66204=ORIENTED_EDGE('',*,*,#50150,.T.);
#66205=ORIENTED_EDGE('',*,*,#48503,.F.);
#66206=ORIENTED_EDGE('',*,*,#50151,.T.);
#66207=ORIENTED_EDGE('',*,*,#48507,.F.);
#66208=ORIENTED_EDGE('',*,*,#50152,.T.);
#66209=ORIENTED_EDGE('',*,*,#48547,.F.);
#66210=ORIENTED_EDGE('',*,*,#50153,.T.);
#66211=ORIENTED_EDGE('',*,*,#48529,.F.);
#66212=ORIENTED_EDGE('',*,*,#50154,.T.);
#66213=ORIENTED_EDGE('',*,*,#48531,.F.);
#66214=ORIENTED_EDGE('',*,*,#50155,.T.);
#66215=ORIENTED_EDGE('',*,*,#48535,.F.);
#66216=ORIENTED_EDGE('',*,*,#50156,.T.);
#66217=ORIENTED_EDGE('',*,*,#48575,.F.);
#66218=ORIENTED_EDGE('',*,*,#50157,.T.);
#66219=ORIENTED_EDGE('',*,*,#48557,.F.);
#66220=ORIENTED_EDGE('',*,*,#50158,.T.);
#66221=ORIENTED_EDGE('',*,*,#48559,.F.);
#66222=ORIENTED_EDGE('',*,*,#50159,.T.);
#66223=ORIENTED_EDGE('',*,*,#48563,.F.);
#66224=ORIENTED_EDGE('',*,*,#50160,.T.);
#66225=ORIENTED_EDGE('',*,*,#48603,.F.);
#66226=ORIENTED_EDGE('',*,*,#50161,.T.);
#66227=ORIENTED_EDGE('',*,*,#48585,.F.);
#66228=ORIENTED_EDGE('',*,*,#50162,.T.);
#66229=ORIENTED_EDGE('',*,*,#48587,.F.);
#66230=ORIENTED_EDGE('',*,*,#50163,.T.);
#66231=ORIENTED_EDGE('',*,*,#48591,.F.);
#66232=ORIENTED_EDGE('',*,*,#50164,.T.);
#66233=ORIENTED_EDGE('',*,*,#48631,.F.);
#66234=ORIENTED_EDGE('',*,*,#50165,.T.);
#66235=ORIENTED_EDGE('',*,*,#48613,.F.);
#66236=ORIENTED_EDGE('',*,*,#50166,.T.);
#66237=ORIENTED_EDGE('',*,*,#48615,.F.);
#66238=ORIENTED_EDGE('',*,*,#50167,.T.);
#66239=ORIENTED_EDGE('',*,*,#48619,.F.);
#66240=ORIENTED_EDGE('',*,*,#50168,.T.);
#66241=ORIENTED_EDGE('',*,*,#48659,.F.);
#66242=ORIENTED_EDGE('',*,*,#50169,.T.);
#66243=ORIENTED_EDGE('',*,*,#48641,.F.);
#66244=ORIENTED_EDGE('',*,*,#50170,.T.);
#66245=ORIENTED_EDGE('',*,*,#48643,.F.);
#66246=ORIENTED_EDGE('',*,*,#50171,.T.);
#66247=ORIENTED_EDGE('',*,*,#48647,.F.);
#66248=ORIENTED_EDGE('',*,*,#50172,.T.);
#66249=ORIENTED_EDGE('',*,*,#48687,.F.);
#66250=ORIENTED_EDGE('',*,*,#50173,.T.);
#66251=ORIENTED_EDGE('',*,*,#48669,.F.);
#66252=ORIENTED_EDGE('',*,*,#50174,.T.);
#66253=ORIENTED_EDGE('',*,*,#48671,.F.);
#66254=ORIENTED_EDGE('',*,*,#50175,.T.);
#66255=ORIENTED_EDGE('',*,*,#48675,.F.);
#66256=ORIENTED_EDGE('',*,*,#50176,.T.);
#66257=ORIENTED_EDGE('',*,*,#48715,.F.);
#66258=ORIENTED_EDGE('',*,*,#50177,.T.);
#66259=ORIENTED_EDGE('',*,*,#48697,.F.);
#66260=ORIENTED_EDGE('',*,*,#50178,.T.);
#66261=ORIENTED_EDGE('',*,*,#48699,.F.);
#66262=ORIENTED_EDGE('',*,*,#50179,.T.);
#66263=ORIENTED_EDGE('',*,*,#48703,.F.);
#66264=ORIENTED_EDGE('',*,*,#50180,.T.);
#66265=ORIENTED_EDGE('',*,*,#48743,.F.);
#66266=ORIENTED_EDGE('',*,*,#50181,.T.);
#66267=ORIENTED_EDGE('',*,*,#48725,.F.);
#66268=ORIENTED_EDGE('',*,*,#50182,.T.);
#66269=ORIENTED_EDGE('',*,*,#48727,.F.);
#66270=ORIENTED_EDGE('',*,*,#50183,.T.);
#66271=ORIENTED_EDGE('',*,*,#48731,.F.);
#66272=ORIENTED_EDGE('',*,*,#50184,.T.);
#66273=ORIENTED_EDGE('',*,*,#48771,.F.);
#66274=ORIENTED_EDGE('',*,*,#50185,.T.);
#66275=ORIENTED_EDGE('',*,*,#48753,.F.);
#66276=ORIENTED_EDGE('',*,*,#50186,.T.);
#66277=ORIENTED_EDGE('',*,*,#48755,.F.);
#66278=ORIENTED_EDGE('',*,*,#50187,.T.);
#66279=ORIENTED_EDGE('',*,*,#48759,.F.);
#66280=ORIENTED_EDGE('',*,*,#50188,.T.);
#66281=ORIENTED_EDGE('',*,*,#48799,.F.);
#66282=ORIENTED_EDGE('',*,*,#50189,.T.);
#66283=ORIENTED_EDGE('',*,*,#48781,.F.);
#66284=ORIENTED_EDGE('',*,*,#50190,.T.);
#66285=ORIENTED_EDGE('',*,*,#48783,.F.);
#66286=ORIENTED_EDGE('',*,*,#50191,.T.);
#66287=ORIENTED_EDGE('',*,*,#48787,.F.);
#66288=ORIENTED_EDGE('',*,*,#50192,.T.);
#66289=ORIENTED_EDGE('',*,*,#48827,.F.);
#66290=ORIENTED_EDGE('',*,*,#50193,.T.);
#66291=ORIENTED_EDGE('',*,*,#48809,.F.);
#66292=ORIENTED_EDGE('',*,*,#50194,.T.);
#66293=ORIENTED_EDGE('',*,*,#48811,.F.);
#66294=ORIENTED_EDGE('',*,*,#50195,.T.);
#66295=ORIENTED_EDGE('',*,*,#48815,.F.);
#66296=ORIENTED_EDGE('',*,*,#50196,.T.);
#66297=ORIENTED_EDGE('',*,*,#48855,.F.);
#66298=ORIENTED_EDGE('',*,*,#50197,.T.);
#66299=ORIENTED_EDGE('',*,*,#48837,.F.);
#66300=ORIENTED_EDGE('',*,*,#50198,.T.);
#66301=ORIENTED_EDGE('',*,*,#48839,.F.);
#66302=ORIENTED_EDGE('',*,*,#50199,.T.);
#66303=ORIENTED_EDGE('',*,*,#48843,.F.);
#66304=ORIENTED_EDGE('',*,*,#50200,.T.);
#66305=ORIENTED_EDGE('',*,*,#48883,.F.);
#66306=ORIENTED_EDGE('',*,*,#50201,.T.);
#66307=ORIENTED_EDGE('',*,*,#48865,.F.);
#66308=ORIENTED_EDGE('',*,*,#50202,.T.);
#66309=ORIENTED_EDGE('',*,*,#48867,.F.);
#66310=ORIENTED_EDGE('',*,*,#50203,.T.);
#66311=ORIENTED_EDGE('',*,*,#48871,.F.);
#66312=ORIENTED_EDGE('',*,*,#50204,.T.);
#66313=ORIENTED_EDGE('',*,*,#48911,.F.);
#66314=ORIENTED_EDGE('',*,*,#50205,.T.);
#66315=ORIENTED_EDGE('',*,*,#48893,.F.);
#66316=ORIENTED_EDGE('',*,*,#50206,.T.);
#66317=ORIENTED_EDGE('',*,*,#48895,.F.);
#66318=ORIENTED_EDGE('',*,*,#50207,.T.);
#66319=ORIENTED_EDGE('',*,*,#48899,.F.);
#66320=ORIENTED_EDGE('',*,*,#50208,.T.);
#66321=ORIENTED_EDGE('',*,*,#48939,.F.);
#66322=ORIENTED_EDGE('',*,*,#50209,.T.);
#66323=ORIENTED_EDGE('',*,*,#48921,.F.);
#66324=ORIENTED_EDGE('',*,*,#50210,.T.);
#66325=ORIENTED_EDGE('',*,*,#48923,.F.);
#66326=ORIENTED_EDGE('',*,*,#50211,.T.);
#66327=ORIENTED_EDGE('',*,*,#48927,.F.);
#66328=ORIENTED_EDGE('',*,*,#50212,.T.);
#66329=ORIENTED_EDGE('',*,*,#48967,.F.);
#66330=ORIENTED_EDGE('',*,*,#50213,.T.);
#66331=ORIENTED_EDGE('',*,*,#48949,.F.);
#66332=ORIENTED_EDGE('',*,*,#50214,.T.);
#66333=ORIENTED_EDGE('',*,*,#48951,.F.);
#66334=ORIENTED_EDGE('',*,*,#50215,.T.);
#66335=ORIENTED_EDGE('',*,*,#48955,.F.);
#66336=ORIENTED_EDGE('',*,*,#50216,.T.);
#66337=ORIENTED_EDGE('',*,*,#48995,.F.);
#66338=ORIENTED_EDGE('',*,*,#50217,.T.);
#66339=ORIENTED_EDGE('',*,*,#48977,.F.);
#66340=ORIENTED_EDGE('',*,*,#50218,.T.);
#66341=ORIENTED_EDGE('',*,*,#48979,.F.);
#66342=ORIENTED_EDGE('',*,*,#50219,.T.);
#66343=ORIENTED_EDGE('',*,*,#48983,.F.);
#66344=ORIENTED_EDGE('',*,*,#50220,.T.);
#66345=ORIENTED_EDGE('',*,*,#49023,.F.);
#66346=ORIENTED_EDGE('',*,*,#50221,.T.);
#66347=ORIENTED_EDGE('',*,*,#49005,.F.);
#66348=ORIENTED_EDGE('',*,*,#50222,.T.);
#66349=ORIENTED_EDGE('',*,*,#49007,.F.);
#66350=ORIENTED_EDGE('',*,*,#50223,.T.);
#66351=ORIENTED_EDGE('',*,*,#49011,.F.);
#66352=ORIENTED_EDGE('',*,*,#50224,.T.);
#66353=ORIENTED_EDGE('',*,*,#49051,.F.);
#66354=ORIENTED_EDGE('',*,*,#50225,.T.);
#66355=ORIENTED_EDGE('',*,*,#49033,.F.);
#66356=ORIENTED_EDGE('',*,*,#50226,.T.);
#66357=ORIENTED_EDGE('',*,*,#49035,.F.);
#66358=ORIENTED_EDGE('',*,*,#50227,.T.);
#66359=ORIENTED_EDGE('',*,*,#49039,.F.);
#66360=ORIENTED_EDGE('',*,*,#50228,.T.);
#66361=ORIENTED_EDGE('',*,*,#49079,.F.);
#66362=ORIENTED_EDGE('',*,*,#50229,.T.);
#66363=ORIENTED_EDGE('',*,*,#49061,.F.);
#66364=ORIENTED_EDGE('',*,*,#50230,.T.);
#66365=ORIENTED_EDGE('',*,*,#49063,.F.);
#66366=ORIENTED_EDGE('',*,*,#50231,.T.);
#66367=ORIENTED_EDGE('',*,*,#49067,.F.);
#66368=ORIENTED_EDGE('',*,*,#50232,.T.);
#66369=ORIENTED_EDGE('',*,*,#49107,.F.);
#66370=ORIENTED_EDGE('',*,*,#50233,.T.);
#66371=ORIENTED_EDGE('',*,*,#49089,.F.);
#66372=ORIENTED_EDGE('',*,*,#50234,.T.);
#66373=ORIENTED_EDGE('',*,*,#49091,.F.);
#66374=ORIENTED_EDGE('',*,*,#50235,.T.);
#66375=ORIENTED_EDGE('',*,*,#49095,.F.);
#66376=ORIENTED_EDGE('',*,*,#50236,.T.);
#66377=ORIENTED_EDGE('',*,*,#49135,.F.);
#66378=ORIENTED_EDGE('',*,*,#50237,.T.);
#66379=ORIENTED_EDGE('',*,*,#49117,.F.);
#66380=ORIENTED_EDGE('',*,*,#50238,.T.);
#66381=ORIENTED_EDGE('',*,*,#49119,.F.);
#66382=ORIENTED_EDGE('',*,*,#50239,.T.);
#66383=ORIENTED_EDGE('',*,*,#49123,.F.);
#66384=ORIENTED_EDGE('',*,*,#50240,.T.);
#66385=ORIENTED_EDGE('',*,*,#49163,.F.);
#66386=ORIENTED_EDGE('',*,*,#50241,.T.);
#66387=ORIENTED_EDGE('',*,*,#49145,.F.);
#66388=ORIENTED_EDGE('',*,*,#50242,.T.);
#66389=ORIENTED_EDGE('',*,*,#49147,.F.);
#66390=ORIENTED_EDGE('',*,*,#50243,.T.);
#66391=ORIENTED_EDGE('',*,*,#49151,.F.);
#66392=ORIENTED_EDGE('',*,*,#50244,.T.);
#66393=ORIENTED_EDGE('',*,*,#49191,.F.);
#66394=ORIENTED_EDGE('',*,*,#50245,.T.);
#66395=ORIENTED_EDGE('',*,*,#49173,.F.);
#66396=ORIENTED_EDGE('',*,*,#50246,.T.);
#66397=ORIENTED_EDGE('',*,*,#49175,.F.);
#66398=ORIENTED_EDGE('',*,*,#50247,.T.);
#66399=ORIENTED_EDGE('',*,*,#49179,.F.);
#66400=ORIENTED_EDGE('',*,*,#50248,.T.);
#66401=ORIENTED_EDGE('',*,*,#49219,.F.);
#66402=ORIENTED_EDGE('',*,*,#50249,.T.);
#66403=ORIENTED_EDGE('',*,*,#49201,.F.);
#66404=ORIENTED_EDGE('',*,*,#50250,.T.);
#66405=ORIENTED_EDGE('',*,*,#49203,.F.);
#66406=ORIENTED_EDGE('',*,*,#50251,.T.);
#66407=ORIENTED_EDGE('',*,*,#49207,.F.);
#66408=ORIENTED_EDGE('',*,*,#50252,.T.);
#66409=ORIENTED_EDGE('',*,*,#49247,.F.);
#66410=ORIENTED_EDGE('',*,*,#50253,.T.);
#66411=ORIENTED_EDGE('',*,*,#49229,.F.);
#66412=ORIENTED_EDGE('',*,*,#50254,.T.);
#66413=ORIENTED_EDGE('',*,*,#49231,.F.);
#66414=ORIENTED_EDGE('',*,*,#50255,.T.);
#66415=ORIENTED_EDGE('',*,*,#49235,.F.);
#66416=ORIENTED_EDGE('',*,*,#50256,.T.);
#66417=ORIENTED_EDGE('',*,*,#49275,.F.);
#66418=ORIENTED_EDGE('',*,*,#50257,.T.);
#66419=ORIENTED_EDGE('',*,*,#49257,.F.);
#66420=ORIENTED_EDGE('',*,*,#50258,.T.);
#66421=ORIENTED_EDGE('',*,*,#49259,.F.);
#66422=ORIENTED_EDGE('',*,*,#50259,.T.);
#66423=ORIENTED_EDGE('',*,*,#49263,.F.);
#66424=ORIENTED_EDGE('',*,*,#50260,.T.);
#66425=ORIENTED_EDGE('',*,*,#49303,.F.);
#66426=ORIENTED_EDGE('',*,*,#50261,.T.);
#66427=ORIENTED_EDGE('',*,*,#49285,.F.);
#66428=ORIENTED_EDGE('',*,*,#50262,.T.);
#66429=ORIENTED_EDGE('',*,*,#49287,.F.);
#66430=ORIENTED_EDGE('',*,*,#50263,.T.);
#66431=ORIENTED_EDGE('',*,*,#49291,.F.);
#66432=ORIENTED_EDGE('',*,*,#50264,.T.);
#66433=ORIENTED_EDGE('',*,*,#49329,.F.);
#66434=ORIENTED_EDGE('',*,*,#50265,.T.);
#66435=ORIENTED_EDGE('',*,*,#49313,.F.);
#66436=ORIENTED_EDGE('',*,*,#50266,.T.);
#66437=ORIENTED_EDGE('',*,*,#49314,.F.);
#66438=ORIENTED_EDGE('',*,*,#50267,.T.);
#66439=ORIENTED_EDGE('',*,*,#49317,.F.);
#66440=ORIENTED_EDGE('',*,*,#50268,.T.);
#66441=ORIENTED_EDGE('',*,*,#49357,.F.);
#66442=ORIENTED_EDGE('',*,*,#50269,.T.);
#66443=ORIENTED_EDGE('',*,*,#49339,.F.);
#66444=ORIENTED_EDGE('',*,*,#50270,.T.);
#66445=ORIENTED_EDGE('',*,*,#49341,.F.);
#66446=ORIENTED_EDGE('',*,*,#50271,.T.);
#66447=ORIENTED_EDGE('',*,*,#49345,.F.);
#66448=ORIENTED_EDGE('',*,*,#50272,.T.);
#66449=ORIENTED_EDGE('',*,*,#49385,.F.);
#66450=ORIENTED_EDGE('',*,*,#50273,.T.);
#66451=ORIENTED_EDGE('',*,*,#49367,.F.);
#66452=ORIENTED_EDGE('',*,*,#50274,.T.);
#66453=ORIENTED_EDGE('',*,*,#49369,.F.);
#66454=ORIENTED_EDGE('',*,*,#50275,.T.);
#66455=ORIENTED_EDGE('',*,*,#49373,.F.);
#66456=ORIENTED_EDGE('',*,*,#50276,.T.);
#66457=ORIENTED_EDGE('',*,*,#49413,.F.);
#66458=ORIENTED_EDGE('',*,*,#50277,.T.);
#66459=ORIENTED_EDGE('',*,*,#49395,.F.);
#66460=ORIENTED_EDGE('',*,*,#50278,.T.);
#66461=ORIENTED_EDGE('',*,*,#49397,.F.);
#66462=ORIENTED_EDGE('',*,*,#50279,.T.);
#66463=ORIENTED_EDGE('',*,*,#49401,.F.);
#66464=ORIENTED_EDGE('',*,*,#50280,.T.);
#66465=ORIENTED_EDGE('',*,*,#49441,.F.);
#66466=ORIENTED_EDGE('',*,*,#50281,.T.);
#66467=ORIENTED_EDGE('',*,*,#49423,.F.);
#66468=ORIENTED_EDGE('',*,*,#50282,.T.);
#66469=ORIENTED_EDGE('',*,*,#49425,.F.);
#66470=ORIENTED_EDGE('',*,*,#50283,.T.);
#66471=ORIENTED_EDGE('',*,*,#49429,.F.);
#66472=ORIENTED_EDGE('',*,*,#50284,.T.);
#66473=ORIENTED_EDGE('',*,*,#49469,.F.);
#66474=ORIENTED_EDGE('',*,*,#50285,.T.);
#66475=ORIENTED_EDGE('',*,*,#49451,.F.);
#66476=ORIENTED_EDGE('',*,*,#50286,.T.);
#66477=ORIENTED_EDGE('',*,*,#49453,.F.);
#66478=ORIENTED_EDGE('',*,*,#50287,.T.);
#66479=ORIENTED_EDGE('',*,*,#49457,.F.);
#66480=ORIENTED_EDGE('',*,*,#50288,.T.);
#66481=ORIENTED_EDGE('',*,*,#49497,.F.);
#66482=ORIENTED_EDGE('',*,*,#50289,.T.);
#66483=ORIENTED_EDGE('',*,*,#49479,.F.);
#66484=ORIENTED_EDGE('',*,*,#50290,.T.);
#66485=ORIENTED_EDGE('',*,*,#49481,.F.);
#66486=ORIENTED_EDGE('',*,*,#50291,.T.);
#66487=ORIENTED_EDGE('',*,*,#49485,.F.);
#66488=ORIENTED_EDGE('',*,*,#50292,.T.);
#66489=ORIENTED_EDGE('',*,*,#49525,.F.);
#66490=ORIENTED_EDGE('',*,*,#50293,.T.);
#66491=ORIENTED_EDGE('',*,*,#49507,.F.);
#66492=ORIENTED_EDGE('',*,*,#50294,.T.);
#66493=ORIENTED_EDGE('',*,*,#49509,.F.);
#66494=ORIENTED_EDGE('',*,*,#50295,.T.);
#66495=ORIENTED_EDGE('',*,*,#49513,.F.);
#66496=ORIENTED_EDGE('',*,*,#50296,.T.);
#66497=ORIENTED_EDGE('',*,*,#49553,.F.);
#66498=ORIENTED_EDGE('',*,*,#50297,.T.);
#66499=ORIENTED_EDGE('',*,*,#49535,.F.);
#66500=ORIENTED_EDGE('',*,*,#50298,.T.);
#66501=ORIENTED_EDGE('',*,*,#49537,.F.);
#66502=ORIENTED_EDGE('',*,*,#50299,.T.);
#66503=ORIENTED_EDGE('',*,*,#49541,.F.);
#66504=ORIENTED_EDGE('',*,*,#50300,.T.);
#66505=ORIENTED_EDGE('',*,*,#49581,.F.);
#66506=ORIENTED_EDGE('',*,*,#50301,.T.);
#66507=ORIENTED_EDGE('',*,*,#49563,.F.);
#66508=ORIENTED_EDGE('',*,*,#50302,.T.);
#66509=ORIENTED_EDGE('',*,*,#49565,.F.);
#66510=ORIENTED_EDGE('',*,*,#50303,.T.);
#66511=ORIENTED_EDGE('',*,*,#49569,.F.);
#66512=ORIENTED_EDGE('',*,*,#50304,.T.);
#66513=ORIENTED_EDGE('',*,*,#49609,.F.);
#66514=ORIENTED_EDGE('',*,*,#50305,.T.);
#66515=ORIENTED_EDGE('',*,*,#49591,.F.);
#66516=ORIENTED_EDGE('',*,*,#50306,.T.);
#66517=ORIENTED_EDGE('',*,*,#49593,.F.);
#66518=ORIENTED_EDGE('',*,*,#50307,.T.);
#66519=ORIENTED_EDGE('',*,*,#49597,.F.);
#66520=ORIENTED_EDGE('',*,*,#50308,.T.);
#66521=ORIENTED_EDGE('',*,*,#49637,.F.);
#66522=ORIENTED_EDGE('',*,*,#50309,.T.);
#66523=ORIENTED_EDGE('',*,*,#49619,.F.);
#66524=ORIENTED_EDGE('',*,*,#50310,.T.);
#66525=ORIENTED_EDGE('',*,*,#49621,.F.);
#66526=ORIENTED_EDGE('',*,*,#50311,.T.);
#66527=ORIENTED_EDGE('',*,*,#49625,.F.);
#66528=ORIENTED_EDGE('',*,*,#50312,.T.);
#66529=ORIENTED_EDGE('',*,*,#49665,.F.);
#66530=ORIENTED_EDGE('',*,*,#50313,.T.);
#66531=ORIENTED_EDGE('',*,*,#49647,.F.);
#66532=ORIENTED_EDGE('',*,*,#50314,.T.);
#66533=ORIENTED_EDGE('',*,*,#49649,.F.);
#66534=ORIENTED_EDGE('',*,*,#50315,.T.);
#66535=ORIENTED_EDGE('',*,*,#49653,.F.);
#66536=ORIENTED_EDGE('',*,*,#50316,.T.);
#66537=ORIENTED_EDGE('',*,*,#49693,.F.);
#66538=ORIENTED_EDGE('',*,*,#50317,.T.);
#66539=ORIENTED_EDGE('',*,*,#49675,.F.);
#66540=ORIENTED_EDGE('',*,*,#50318,.T.);
#66541=ORIENTED_EDGE('',*,*,#49677,.F.);
#66542=ORIENTED_EDGE('',*,*,#50319,.T.);
#66543=ORIENTED_EDGE('',*,*,#49681,.F.);
#66544=ORIENTED_EDGE('',*,*,#50320,.T.);
#66545=ORIENTED_EDGE('',*,*,#49721,.F.);
#66546=ORIENTED_EDGE('',*,*,#50321,.T.);
#66547=ORIENTED_EDGE('',*,*,#49703,.F.);
#66548=ORIENTED_EDGE('',*,*,#50322,.T.);
#66549=ORIENTED_EDGE('',*,*,#49705,.F.);
#66550=ORIENTED_EDGE('',*,*,#50323,.T.);
#66551=ORIENTED_EDGE('',*,*,#49709,.F.);
#66552=ORIENTED_EDGE('',*,*,#50324,.T.);
#66553=ORIENTED_EDGE('',*,*,#49747,.F.);
#66554=ORIENTED_EDGE('',*,*,#50325,.T.);
#66555=ORIENTED_EDGE('',*,*,#49731,.F.);
#66556=ORIENTED_EDGE('',*,*,#50326,.T.);
#66557=ORIENTED_EDGE('',*,*,#49732,.F.);
#66558=ORIENTED_EDGE('',*,*,#50327,.T.);
#66559=ORIENTED_EDGE('',*,*,#49735,.F.);
#66560=ORIENTED_EDGE('',*,*,#50328,.T.);
#66561=ORIENTED_EDGE('',*,*,#49775,.F.);
#66562=ORIENTED_EDGE('',*,*,#50329,.T.);
#66563=ORIENTED_EDGE('',*,*,#49757,.F.);
#66564=ORIENTED_EDGE('',*,*,#50330,.T.);
#66565=ORIENTED_EDGE('',*,*,#49759,.F.);
#66566=ORIENTED_EDGE('',*,*,#50331,.T.);
#66567=ORIENTED_EDGE('',*,*,#49763,.F.);
#66568=ORIENTED_EDGE('',*,*,#50332,.T.);
#66569=ORIENTED_EDGE('',*,*,#49803,.F.);
#66570=ORIENTED_EDGE('',*,*,#50333,.T.);
#66571=ORIENTED_EDGE('',*,*,#49785,.F.);
#66572=ORIENTED_EDGE('',*,*,#50334,.T.);
#66573=ORIENTED_EDGE('',*,*,#49787,.F.);
#66574=ORIENTED_EDGE('',*,*,#50335,.T.);
#66575=ORIENTED_EDGE('',*,*,#49791,.F.);
#66576=ORIENTED_EDGE('',*,*,#50336,.T.);
#66577=ORIENTED_EDGE('',*,*,#49831,.F.);
#66578=ORIENTED_EDGE('',*,*,#50337,.T.);
#66579=ORIENTED_EDGE('',*,*,#49813,.F.);
#66580=ORIENTED_EDGE('',*,*,#50338,.T.);
#66581=ORIENTED_EDGE('',*,*,#49815,.F.);
#66582=ORIENTED_EDGE('',*,*,#50339,.T.);
#66583=ORIENTED_EDGE('',*,*,#49819,.F.);
#66584=ORIENTED_EDGE('',*,*,#50340,.T.);
#66585=ORIENTED_EDGE('',*,*,#49859,.F.);
#66586=ORIENTED_EDGE('',*,*,#50341,.T.);
#66587=ORIENTED_EDGE('',*,*,#49841,.F.);
#66588=ORIENTED_EDGE('',*,*,#50342,.T.);
#66589=ORIENTED_EDGE('',*,*,#49843,.F.);
#66590=ORIENTED_EDGE('',*,*,#50343,.T.);
#66591=ORIENTED_EDGE('',*,*,#49847,.F.);
#66592=ORIENTED_EDGE('',*,*,#50344,.T.);
#66593=ORIENTED_EDGE('',*,*,#49887,.F.);
#66594=ORIENTED_EDGE('',*,*,#50345,.T.);
#66595=ORIENTED_EDGE('',*,*,#49869,.F.);
#66596=ORIENTED_EDGE('',*,*,#50346,.T.);
#66597=ORIENTED_EDGE('',*,*,#49871,.F.);
#66598=ORIENTED_EDGE('',*,*,#50347,.T.);
#66599=ORIENTED_EDGE('',*,*,#49875,.F.);
#66600=ORIENTED_EDGE('',*,*,#50348,.T.);
#66601=ORIENTED_EDGE('',*,*,#49915,.F.);
#66602=ORIENTED_EDGE('',*,*,#50349,.T.);
#66603=ORIENTED_EDGE('',*,*,#49897,.F.);
#66604=ORIENTED_EDGE('',*,*,#50350,.T.);
#66605=ORIENTED_EDGE('',*,*,#49899,.F.);
#66606=ORIENTED_EDGE('',*,*,#50351,.T.);
#66607=ORIENTED_EDGE('',*,*,#49903,.F.);
#66608=ORIENTED_EDGE('',*,*,#50352,.T.);
#66609=ORIENTED_EDGE('',*,*,#49943,.F.);
#66610=ORIENTED_EDGE('',*,*,#50353,.T.);
#66611=ORIENTED_EDGE('',*,*,#49925,.F.);
#66612=ORIENTED_EDGE('',*,*,#50354,.T.);
#66613=ORIENTED_EDGE('',*,*,#49927,.F.);
#66614=ORIENTED_EDGE('',*,*,#50355,.T.);
#66615=ORIENTED_EDGE('',*,*,#49931,.F.);
#66616=ORIENTED_EDGE('',*,*,#50356,.T.);
#66617=ORIENTED_EDGE('',*,*,#49971,.F.);
#66618=ORIENTED_EDGE('',*,*,#50357,.T.);
#66619=ORIENTED_EDGE('',*,*,#49953,.F.);
#66620=ORIENTED_EDGE('',*,*,#50358,.T.);
#66621=ORIENTED_EDGE('',*,*,#49955,.F.);
#66622=ORIENTED_EDGE('',*,*,#50359,.T.);
#66623=ORIENTED_EDGE('',*,*,#49959,.F.);
#66624=ORIENTED_EDGE('',*,*,#50360,.T.);
#66625=ORIENTED_EDGE('',*,*,#49999,.F.);
#66626=ORIENTED_EDGE('',*,*,#50361,.T.);
#66627=ORIENTED_EDGE('',*,*,#49981,.F.);
#66628=ORIENTED_EDGE('',*,*,#50362,.T.);
#66629=ORIENTED_EDGE('',*,*,#49983,.F.);
#66630=ORIENTED_EDGE('',*,*,#50363,.T.);
#66631=ORIENTED_EDGE('',*,*,#49987,.F.);
#66632=ORIENTED_EDGE('',*,*,#50364,.T.);
#66633=ORIENTED_EDGE('',*,*,#50027,.F.);
#66634=ORIENTED_EDGE('',*,*,#50365,.T.);
#66635=ORIENTED_EDGE('',*,*,#50009,.F.);
#66636=ORIENTED_EDGE('',*,*,#50366,.T.);
#66637=ORIENTED_EDGE('',*,*,#50011,.F.);
#66638=ORIENTED_EDGE('',*,*,#50367,.T.);
#66639=ORIENTED_EDGE('',*,*,#50015,.F.);
#66640=ORIENTED_EDGE('',*,*,#50368,.T.);
#66641=ORIENTED_EDGE('',*,*,#50055,.F.);
#66642=ORIENTED_EDGE('',*,*,#50369,.T.);
#66643=ORIENTED_EDGE('',*,*,#50037,.F.);
#66644=ORIENTED_EDGE('',*,*,#50370,.T.);
#66645=ORIENTED_EDGE('',*,*,#50039,.F.);
#66646=ORIENTED_EDGE('',*,*,#50371,.T.);
#66647=ORIENTED_EDGE('',*,*,#50043,.F.);
#66648=ORIENTED_EDGE('',*,*,#50372,.T.);
#66649=ORIENTED_EDGE('',*,*,#50083,.F.);
#66650=ORIENTED_EDGE('',*,*,#50373,.T.);
#66651=ORIENTED_EDGE('',*,*,#50065,.F.);
#66652=ORIENTED_EDGE('',*,*,#50374,.T.);
#66653=ORIENTED_EDGE('',*,*,#50067,.F.);
#66654=ORIENTED_EDGE('',*,*,#50375,.T.);
#66655=ORIENTED_EDGE('',*,*,#50071,.F.);
#66656=ORIENTED_EDGE('',*,*,#50376,.T.);
#66657=ORIENTED_EDGE('',*,*,#50111,.F.);
#66658=ORIENTED_EDGE('',*,*,#50377,.T.);
#66659=ORIENTED_EDGE('',*,*,#50093,.F.);
#66660=ORIENTED_EDGE('',*,*,#50378,.T.);
#66661=ORIENTED_EDGE('',*,*,#50095,.F.);
#66662=ORIENTED_EDGE('',*,*,#50379,.T.);
#66663=ORIENTED_EDGE('',*,*,#50099,.F.);
#66664=ORIENTED_EDGE('',*,*,#50380,.T.);
#66665=ORIENTED_EDGE('',*,*,#50139,.F.);
#66666=ORIENTED_EDGE('',*,*,#50381,.T.);
#66667=ORIENTED_EDGE('',*,*,#50121,.F.);
#66668=ORIENTED_EDGE('',*,*,#50382,.T.);
#66669=ORIENTED_EDGE('',*,*,#50123,.F.);
#66670=ORIENTED_EDGE('',*,*,#50383,.T.);
#66671=ORIENTED_EDGE('',*,*,#50127,.F.);
#66672=ORIENTED_EDGE('',*,*,#50384,.T.);
#66673=ORIENTED_EDGE('',*,*,#50385,.F.);
#66674=ORIENTED_EDGE('',*,*,#48527,.F.);
#66675=ORIENTED_EDGE('',*,*,#50386,.F.);
#66676=ORIENTED_EDGE('',*,*,#48399,.F.);
#66677=ORIENTED_EDGE('',*,*,#50386,.T.);
#66678=ORIENTED_EDGE('',*,*,#48526,.F.);
#66679=ORIENTED_EDGE('',*,*,#50387,.F.);
#66680=ORIENTED_EDGE('',*,*,#48408,.F.);
#66681=ORIENTED_EDGE('',*,*,#48398,.T.);
#66682=ORIENTED_EDGE('',*,*,#48402,.F.);
#66683=ORIENTED_EDGE('',*,*,#50388,.F.);
#66684=ORIENTED_EDGE('',*,*,#48528,.F.);
#66685=ORIENTED_EDGE('',*,*,#50385,.T.);
#66686=ORIENTED_EDGE('',*,*,#50387,.T.);
#66687=ORIENTED_EDGE('',*,*,#48525,.F.);
#66688=ORIENTED_EDGE('',*,*,#50389,.F.);
#66689=ORIENTED_EDGE('',*,*,#48393,.F.);
#66690=ORIENTED_EDGE('',*,*,#50388,.T.);
#66691=ORIENTED_EDGE('',*,*,#48406,.F.);
#66692=ORIENTED_EDGE('',*,*,#50390,.F.);
#66693=ORIENTED_EDGE('',*,*,#48517,.F.);
#66694=ORIENTED_EDGE('',*,*,#50389,.T.);
#66695=ORIENTED_EDGE('',*,*,#48524,.F.);
#66696=ORIENTED_EDGE('',*,*,#50391,.F.);
#66697=ORIENTED_EDGE('',*,*,#48410,.F.);
#66698=ORIENTED_EDGE('',*,*,#50390,.T.);
#66699=ORIENTED_EDGE('',*,*,#45925,.F.);
#66700=ORIENTED_EDGE('',*,*,#50392,.F.);
#66701=ORIENTED_EDGE('',*,*,#48518,.F.);
#66702=ORIENTED_EDGE('',*,*,#50391,.T.);
#66703=ORIENTED_EDGE('',*,*,#48523,.F.);
#66704=ORIENTED_EDGE('',*,*,#50393,.F.);
#66705=ORIENTED_EDGE('',*,*,#48385,.T.);
#66706=ORIENTED_EDGE('',*,*,#48389,.F.);
#66707=ORIENTED_EDGE('',*,*,#50392,.T.);
#66708=ORIENTED_EDGE('',*,*,#45924,.F.);
#66709=ORIENTED_EDGE('',*,*,#50394,.F.);
#66710=ORIENTED_EDGE('',*,*,#50149,.F.);
#66711=ORIENTED_EDGE('',*,*,#50393,.T.);
#66712=ORIENTED_EDGE('',*,*,#48522,.F.);
#66713=ORIENTED_EDGE('',*,*,#50395,.F.);
#66714=ORIENTED_EDGE('',*,*,#48386,.F.);
#66715=ORIENTED_EDGE('',*,*,#50394,.T.);
#66716=ORIENTED_EDGE('',*,*,#45923,.F.);
#66717=ORIENTED_EDGE('',*,*,#50396,.F.);
#66718=ORIENTED_EDGE('',*,*,#48502,.F.);
#66719=ORIENTED_EDGE('',*,*,#50395,.T.);
#66720=ORIENTED_EDGE('',*,*,#48521,.F.);
#66721=ORIENTED_EDGE('',*,*,#50397,.F.);
#66722=ORIENTED_EDGE('',*,*,#48404,.F.);
#66723=ORIENTED_EDGE('',*,*,#50396,.T.);
#66724=ORIENTED_EDGE('',*,*,#45922,.F.);
#66725=ORIENTED_EDGE('',*,*,#50398,.F.);
#66726=ORIENTED_EDGE('',*,*,#50151,.F.);
#66727=ORIENTED_EDGE('',*,*,#50397,.T.);
#66728=ORIENTED_EDGE('',*,*,#48520,.F.);
#66729=ORIENTED_EDGE('',*,*,#50399,.F.);
#66730=ORIENTED_EDGE('',*,*,#46447,.F.);
#66731=ORIENTED_EDGE('',*,*,#50398,.T.);
#66732=ORIENTED_EDGE('',*,*,#45921,.F.);
#66733=ORIENTED_EDGE('',*,*,#50400,.F.);
#66734=ORIENTED_EDGE('',*,*,#48508,.F.);
#66735=ORIENTED_EDGE('',*,*,#50399,.T.);
#66736=ORIENTED_EDGE('',*,*,#50150,.F.);
#66737=ORIENTED_EDGE('',*,*,#50401,.F.);
#66738=ORIENTED_EDGE('',*,*,#46448,.F.);
#66739=ORIENTED_EDGE('',*,*,#50400,.T.);
#66740=ORIENTED_EDGE('',*,*,#48435,.F.);
#66741=ORIENTED_EDGE('',*,*,#50402,.F.);
#66742=ORIENTED_EDGE('',*,*,#48509,.F.);
#66743=ORIENTED_EDGE('',*,*,#50401,.T.);
#66744=ORIENTED_EDGE('',*,*,#48504,.F.);
#66745=ORIENTED_EDGE('',*,*,#50403,.F.);
#66746=ORIENTED_EDGE('',*,*,#46449,.F.);
#66747=ORIENTED_EDGE('',*,*,#48430,.F.);
#66748=ORIENTED_EDGE('',*,*,#48426,.T.);
#66749=ORIENTED_EDGE('',*,*,#50404,.F.);
#66750=ORIENTED_EDGE('',*,*,#48510,.F.);
#66751=ORIENTED_EDGE('',*,*,#50402,.T.);
#66752=ORIENTED_EDGE('',*,*,#50403,.T.);
#66753=ORIENTED_EDGE('',*,*,#50152,.F.);
#66754=ORIENTED_EDGE('',*,*,#50405,.F.);
#66755=ORIENTED_EDGE('',*,*,#46450,.F.);
#66756=ORIENTED_EDGE('',*,*,#50404,.T.);
#66757=ORIENTED_EDGE('',*,*,#48425,.F.);
#66758=ORIENTED_EDGE('',*,*,#50406,.F.);
#66759=ORIENTED_EDGE('',*,*,#48511,.F.);
#66760=ORIENTED_EDGE('',*,*,#50405,.T.);
#66761=ORIENTED_EDGE('',*,*,#48506,.F.);
#66762=ORIENTED_EDGE('',*,*,#50407,.F.);
#66763=ORIENTED_EDGE('',*,*,#46451,.F.);
#66764=ORIENTED_EDGE('',*,*,#50406,.T.);
#66765=ORIENTED_EDGE('',*,*,#48437,.F.);
#66766=ORIENTED_EDGE('',*,*,#50408,.F.);
#66767=ORIENTED_EDGE('',*,*,#48512,.F.);
#66768=ORIENTED_EDGE('',*,*,#50407,.T.);
#66769=ORIENTED_EDGE('',*,*,#48505,.F.);
#66770=ORIENTED_EDGE('',*,*,#50409,.F.);
#66771=ORIENTED_EDGE('',*,*,#48433,.F.);
#66772=ORIENTED_EDGE('',*,*,#50408,.T.);
#66773=ORIENTED_EDGE('',*,*,#48421,.F.);
#66774=ORIENTED_EDGE('',*,*,#50410,.F.);
#66775=ORIENTED_EDGE('',*,*,#48513,.F.);
#66776=ORIENTED_EDGE('',*,*,#50409,.T.);
#66777=ORIENTED_EDGE('',*,*,#48516,.F.);
#66778=ORIENTED_EDGE('',*,*,#50411,.F.);
#66779=ORIENTED_EDGE('',*,*,#48412,.F.);
#66780=ORIENTED_EDGE('',*,*,#50410,.T.);
#66781=ORIENTED_EDGE('',*,*,#48439,.F.);
#66782=ORIENTED_EDGE('',*,*,#50412,.F.);
#66783=ORIENTED_EDGE('',*,*,#48514,.F.);
#66784=ORIENTED_EDGE('',*,*,#50411,.T.);
#66785=ORIENTED_EDGE('',*,*,#48515,.F.);
#66786=ORIENTED_EDGE('',*,*,#50412,.T.);
#66787=ORIENTED_EDGE('',*,*,#48417,.F.);
#66788=ORIENTED_EDGE('',*,*,#48413,.T.);
#66789=ORIENTED_EDGE('',*,*,#50413,.F.);
#66790=ORIENTED_EDGE('',*,*,#48555,.F.);
#66791=ORIENTED_EDGE('',*,*,#50414,.F.);
#66792=ORIENTED_EDGE('',*,*,#48369,.F.);
#66793=ORIENTED_EDGE('',*,*,#50414,.T.);
#66794=ORIENTED_EDGE('',*,*,#48554,.F.);
#66795=ORIENTED_EDGE('',*,*,#50415,.F.);
#66796=ORIENTED_EDGE('',*,*,#48378,.F.);
#66797=ORIENTED_EDGE('',*,*,#48368,.T.);
#66798=ORIENTED_EDGE('',*,*,#48372,.F.);
#66799=ORIENTED_EDGE('',*,*,#50416,.F.);
#66800=ORIENTED_EDGE('',*,*,#48556,.F.);
#66801=ORIENTED_EDGE('',*,*,#50413,.T.);
#66802=ORIENTED_EDGE('',*,*,#50415,.T.);
#66803=ORIENTED_EDGE('',*,*,#48553,.F.);
#66804=ORIENTED_EDGE('',*,*,#50417,.F.);
#66805=ORIENTED_EDGE('',*,*,#48363,.F.);
#66806=ORIENTED_EDGE('',*,*,#50416,.T.);
#66807=ORIENTED_EDGE('',*,*,#48376,.F.);
#66808=ORIENTED_EDGE('',*,*,#50418,.F.);
#66809=ORIENTED_EDGE('',*,*,#48545,.F.);
#66810=ORIENTED_EDGE('',*,*,#50417,.T.);
#66811=ORIENTED_EDGE('',*,*,#48552,.F.);
#66812=ORIENTED_EDGE('',*,*,#50419,.F.);
#66813=ORIENTED_EDGE('',*,*,#48380,.F.);
#66814=ORIENTED_EDGE('',*,*,#50418,.T.);
#66815=ORIENTED_EDGE('',*,*,#45931,.F.);
#66816=ORIENTED_EDGE('',*,*,#50420,.F.);
#66817=ORIENTED_EDGE('',*,*,#48546,.F.);
#66818=ORIENTED_EDGE('',*,*,#50419,.T.);
#66819=ORIENTED_EDGE('',*,*,#48551,.F.);
#66820=ORIENTED_EDGE('',*,*,#50421,.F.);
#66821=ORIENTED_EDGE('',*,*,#48355,.T.);
#66822=ORIENTED_EDGE('',*,*,#48359,.F.);
#66823=ORIENTED_EDGE('',*,*,#50420,.T.);
#66824=ORIENTED_EDGE('',*,*,#45930,.F.);
#66825=ORIENTED_EDGE('',*,*,#50422,.F.);
#66826=ORIENTED_EDGE('',*,*,#50153,.F.);
#66827=ORIENTED_EDGE('',*,*,#50421,.T.);
#66828=ORIENTED_EDGE('',*,*,#48550,.F.);
#66829=ORIENTED_EDGE('',*,*,#50423,.F.);
#66830=ORIENTED_EDGE('',*,*,#48356,.F.);
#66831=ORIENTED_EDGE('',*,*,#50422,.T.);
#66832=ORIENTED_EDGE('',*,*,#45929,.F.);
#66833=ORIENTED_EDGE('',*,*,#50424,.F.);
#66834=ORIENTED_EDGE('',*,*,#48530,.F.);
#66835=ORIENTED_EDGE('',*,*,#50423,.T.);
#66836=ORIENTED_EDGE('',*,*,#48549,.F.);
#66837=ORIENTED_EDGE('',*,*,#50425,.F.);
#66838=ORIENTED_EDGE('',*,*,#48374,.F.);
#66839=ORIENTED_EDGE('',*,*,#50424,.T.);
#66840=ORIENTED_EDGE('',*,*,#45928,.F.);
#66841=ORIENTED_EDGE('',*,*,#50426,.F.);
#66842=ORIENTED_EDGE('',*,*,#50155,.F.);
#66843=ORIENTED_EDGE('',*,*,#50425,.T.);
#66844=ORIENTED_EDGE('',*,*,#48548,.F.);
#66845=ORIENTED_EDGE('',*,*,#50427,.F.);
#66846=ORIENTED_EDGE('',*,*,#46441,.F.);
#66847=ORIENTED_EDGE('',*,*,#50426,.T.);
#66848=ORIENTED_EDGE('',*,*,#45927,.F.);
#66849=ORIENTED_EDGE('',*,*,#50428,.F.);
#66850=ORIENTED_EDGE('',*,*,#48536,.F.);
#66851=ORIENTED_EDGE('',*,*,#50427,.T.);
#66852=ORIENTED_EDGE('',*,*,#50154,.F.);
#66853=ORIENTED_EDGE('',*,*,#50429,.F.);
#66854=ORIENTED_EDGE('',*,*,#46442,.F.);
#66855=ORIENTED_EDGE('',*,*,#50428,.T.);
#66856=ORIENTED_EDGE('',*,*,#48405,.F.);
#66857=ORIENTED_EDGE('',*,*,#50430,.F.);
#66858=ORIENTED_EDGE('',*,*,#48537,.F.);
#66859=ORIENTED_EDGE('',*,*,#50429,.T.);
#66860=ORIENTED_EDGE('',*,*,#48532,.F.);
#66861=ORIENTED_EDGE('',*,*,#50431,.F.);
#66862=ORIENTED_EDGE('',*,*,#46443,.F.);
#66863=ORIENTED_EDGE('',*,*,#48400,.F.);
#66864=ORIENTED_EDGE('',*,*,#48396,.T.);
#66865=ORIENTED_EDGE('',*,*,#50432,.F.);
#66866=ORIENTED_EDGE('',*,*,#48538,.F.);
#66867=ORIENTED_EDGE('',*,*,#50430,.T.);
#66868=ORIENTED_EDGE('',*,*,#50431,.T.);
#66869=ORIENTED_EDGE('',*,*,#50156,.F.);
#66870=ORIENTED_EDGE('',*,*,#50433,.F.);
#66871=ORIENTED_EDGE('',*,*,#46444,.F.);
#66872=ORIENTED_EDGE('',*,*,#50432,.T.);
#66873=ORIENTED_EDGE('',*,*,#48395,.F.);
#66874=ORIENTED_EDGE('',*,*,#50434,.F.);
#66875=ORIENTED_EDGE('',*,*,#48539,.F.);
#66876=ORIENTED_EDGE('',*,*,#50433,.T.);
#66877=ORIENTED_EDGE('',*,*,#48534,.F.);
#66878=ORIENTED_EDGE('',*,*,#50435,.F.);
#66879=ORIENTED_EDGE('',*,*,#46445,.F.);
#66880=ORIENTED_EDGE('',*,*,#50434,.T.);
#66881=ORIENTED_EDGE('',*,*,#48407,.F.);
#66882=ORIENTED_EDGE('',*,*,#50436,.F.);
#66883=ORIENTED_EDGE('',*,*,#48540,.F.);
#66884=ORIENTED_EDGE('',*,*,#50435,.T.);
#66885=ORIENTED_EDGE('',*,*,#48533,.F.);
#66886=ORIENTED_EDGE('',*,*,#50437,.F.);
#66887=ORIENTED_EDGE('',*,*,#48403,.F.);
#66888=ORIENTED_EDGE('',*,*,#50436,.T.);
#66889=ORIENTED_EDGE('',*,*,#48391,.F.);
#66890=ORIENTED_EDGE('',*,*,#50438,.F.);
#66891=ORIENTED_EDGE('',*,*,#48541,.F.);
#66892=ORIENTED_EDGE('',*,*,#50437,.T.);
#66893=ORIENTED_EDGE('',*,*,#48544,.F.);
#66894=ORIENTED_EDGE('',*,*,#50439,.F.);
#66895=ORIENTED_EDGE('',*,*,#48382,.F.);
#66896=ORIENTED_EDGE('',*,*,#50438,.T.);
#66897=ORIENTED_EDGE('',*,*,#48409,.F.);
#66898=ORIENTED_EDGE('',*,*,#50440,.F.);
#66899=ORIENTED_EDGE('',*,*,#48542,.F.);
#66900=ORIENTED_EDGE('',*,*,#50439,.T.);
#66901=ORIENTED_EDGE('',*,*,#48543,.F.);
#66902=ORIENTED_EDGE('',*,*,#50440,.T.);
#66903=ORIENTED_EDGE('',*,*,#48387,.F.);
#66904=ORIENTED_EDGE('',*,*,#48383,.T.);
#66905=ORIENTED_EDGE('',*,*,#50441,.F.);
#66906=ORIENTED_EDGE('',*,*,#48583,.F.);
#66907=ORIENTED_EDGE('',*,*,#50442,.F.);
#66908=ORIENTED_EDGE('',*,*,#48339,.F.);
#66909=ORIENTED_EDGE('',*,*,#50442,.T.);
#66910=ORIENTED_EDGE('',*,*,#48582,.F.);
#66911=ORIENTED_EDGE('',*,*,#50443,.F.);
#66912=ORIENTED_EDGE('',*,*,#48348,.F.);
#66913=ORIENTED_EDGE('',*,*,#48338,.T.);
#66914=ORIENTED_EDGE('',*,*,#48342,.F.);
#66915=ORIENTED_EDGE('',*,*,#50444,.F.);
#66916=ORIENTED_EDGE('',*,*,#48584,.F.);
#66917=ORIENTED_EDGE('',*,*,#50441,.T.);
#66918=ORIENTED_EDGE('',*,*,#50443,.T.);
#66919=ORIENTED_EDGE('',*,*,#48581,.F.);
#66920=ORIENTED_EDGE('',*,*,#50445,.F.);
#66921=ORIENTED_EDGE('',*,*,#48333,.F.);
#66922=ORIENTED_EDGE('',*,*,#50444,.T.);
#66923=ORIENTED_EDGE('',*,*,#48346,.F.);
#66924=ORIENTED_EDGE('',*,*,#50446,.F.);
#66925=ORIENTED_EDGE('',*,*,#48573,.F.);
#66926=ORIENTED_EDGE('',*,*,#50445,.T.);
#66927=ORIENTED_EDGE('',*,*,#48580,.F.);
#66928=ORIENTED_EDGE('',*,*,#50447,.F.);
#66929=ORIENTED_EDGE('',*,*,#48350,.F.);
#66930=ORIENTED_EDGE('',*,*,#50446,.T.);
#66931=ORIENTED_EDGE('',*,*,#45937,.F.);
#66932=ORIENTED_EDGE('',*,*,#50448,.F.);
#66933=ORIENTED_EDGE('',*,*,#48574,.F.);
#66934=ORIENTED_EDGE('',*,*,#50447,.T.);
#66935=ORIENTED_EDGE('',*,*,#48579,.F.);
#66936=ORIENTED_EDGE('',*,*,#50449,.F.);
#66937=ORIENTED_EDGE('',*,*,#48325,.T.);
#66938=ORIENTED_EDGE('',*,*,#48329,.F.);
#66939=ORIENTED_EDGE('',*,*,#50448,.T.);
#66940=ORIENTED_EDGE('',*,*,#45936,.F.);
#66941=ORIENTED_EDGE('',*,*,#50450,.F.);
#66942=ORIENTED_EDGE('',*,*,#50157,.F.);
#66943=ORIENTED_EDGE('',*,*,#50449,.T.);
#66944=ORIENTED_EDGE('',*,*,#48578,.F.);
#66945=ORIENTED_EDGE('',*,*,#50451,.F.);
#66946=ORIENTED_EDGE('',*,*,#48326,.F.);
#66947=ORIENTED_EDGE('',*,*,#50450,.T.);
#66948=ORIENTED_EDGE('',*,*,#45935,.F.);
#66949=ORIENTED_EDGE('',*,*,#50452,.F.);
#66950=ORIENTED_EDGE('',*,*,#48558,.F.);
#66951=ORIENTED_EDGE('',*,*,#50451,.T.);
#66952=ORIENTED_EDGE('',*,*,#48577,.F.);
#66953=ORIENTED_EDGE('',*,*,#50453,.F.);
#66954=ORIENTED_EDGE('',*,*,#48344,.F.);
#66955=ORIENTED_EDGE('',*,*,#50452,.T.);
#66956=ORIENTED_EDGE('',*,*,#45934,.F.);
#66957=ORIENTED_EDGE('',*,*,#50454,.F.);
#66958=ORIENTED_EDGE('',*,*,#50159,.F.);
#66959=ORIENTED_EDGE('',*,*,#50453,.T.);
#66960=ORIENTED_EDGE('',*,*,#48576,.F.);
#66961=ORIENTED_EDGE('',*,*,#50455,.F.);
#66962=ORIENTED_EDGE('',*,*,#46435,.F.);
#66963=ORIENTED_EDGE('',*,*,#50454,.T.);
#66964=ORIENTED_EDGE('',*,*,#45933,.F.);
#66965=ORIENTED_EDGE('',*,*,#50456,.F.);
#66966=ORIENTED_EDGE('',*,*,#48564,.F.);
#66967=ORIENTED_EDGE('',*,*,#50455,.T.);
#66968=ORIENTED_EDGE('',*,*,#50158,.F.);
#66969=ORIENTED_EDGE('',*,*,#50457,.F.);
#66970=ORIENTED_EDGE('',*,*,#46436,.F.);
#66971=ORIENTED_EDGE('',*,*,#50456,.T.);
#66972=ORIENTED_EDGE('',*,*,#48375,.F.);
#66973=ORIENTED_EDGE('',*,*,#50458,.F.);
#66974=ORIENTED_EDGE('',*,*,#48565,.F.);
#66975=ORIENTED_EDGE('',*,*,#50457,.T.);
#66976=ORIENTED_EDGE('',*,*,#48560,.F.);
#66977=ORIENTED_EDGE('',*,*,#50459,.F.);
#66978=ORIENTED_EDGE('',*,*,#46437,.F.);
#66979=ORIENTED_EDGE('',*,*,#48370,.F.);
#66980=ORIENTED_EDGE('',*,*,#48366,.T.);
#66981=ORIENTED_EDGE('',*,*,#50460,.F.);
#66982=ORIENTED_EDGE('',*,*,#48566,.F.);
#66983=ORIENTED_EDGE('',*,*,#50458,.T.);
#66984=ORIENTED_EDGE('',*,*,#50459,.T.);
#66985=ORIENTED_EDGE('',*,*,#50160,.F.);
#66986=ORIENTED_EDGE('',*,*,#50461,.F.);
#66987=ORIENTED_EDGE('',*,*,#46438,.F.);
#66988=ORIENTED_EDGE('',*,*,#50460,.T.);
#66989=ORIENTED_EDGE('',*,*,#48365,.F.);
#66990=ORIENTED_EDGE('',*,*,#50462,.F.);
#66991=ORIENTED_EDGE('',*,*,#48567,.F.);
#66992=ORIENTED_EDGE('',*,*,#50461,.T.);
#66993=ORIENTED_EDGE('',*,*,#48562,.F.);
#66994=ORIENTED_EDGE('',*,*,#50463,.F.);
#66995=ORIENTED_EDGE('',*,*,#46439,.F.);
#66996=ORIENTED_EDGE('',*,*,#50462,.T.);
#66997=ORIENTED_EDGE('',*,*,#48377,.F.);
#66998=ORIENTED_EDGE('',*,*,#50464,.F.);
#66999=ORIENTED_EDGE('',*,*,#48568,.F.);
#67000=ORIENTED_EDGE('',*,*,#50463,.T.);
#67001=ORIENTED_EDGE('',*,*,#48561,.F.);
#67002=ORIENTED_EDGE('',*,*,#50465,.F.);
#67003=ORIENTED_EDGE('',*,*,#48373,.F.);
#67004=ORIENTED_EDGE('',*,*,#50464,.T.);
#67005=ORIENTED_EDGE('',*,*,#48361,.F.);
#67006=ORIENTED_EDGE('',*,*,#50466,.F.);
#67007=ORIENTED_EDGE('',*,*,#48569,.F.);
#67008=ORIENTED_EDGE('',*,*,#50465,.T.);
#67009=ORIENTED_EDGE('',*,*,#48572,.F.);
#67010=ORIENTED_EDGE('',*,*,#50467,.F.);
#67011=ORIENTED_EDGE('',*,*,#48352,.F.);
#67012=ORIENTED_EDGE('',*,*,#50466,.T.);
#67013=ORIENTED_EDGE('',*,*,#48379,.F.);
#67014=ORIENTED_EDGE('',*,*,#50468,.F.);
#67015=ORIENTED_EDGE('',*,*,#48570,.F.);
#67016=ORIENTED_EDGE('',*,*,#50467,.T.);
#67017=ORIENTED_EDGE('',*,*,#48571,.F.);
#67018=ORIENTED_EDGE('',*,*,#50468,.T.);
#67019=ORIENTED_EDGE('',*,*,#48357,.F.);
#67020=ORIENTED_EDGE('',*,*,#48353,.T.);
#67021=ORIENTED_EDGE('',*,*,#50469,.F.);
#67022=ORIENTED_EDGE('',*,*,#48611,.F.);
#67023=ORIENTED_EDGE('',*,*,#50470,.F.);
#67024=ORIENTED_EDGE('',*,*,#48309,.F.);
#67025=ORIENTED_EDGE('',*,*,#50470,.T.);
#67026=ORIENTED_EDGE('',*,*,#48610,.F.);
#67027=ORIENTED_EDGE('',*,*,#50471,.F.);
#67028=ORIENTED_EDGE('',*,*,#48318,.F.);
#67029=ORIENTED_EDGE('',*,*,#48308,.T.);
#67030=ORIENTED_EDGE('',*,*,#48312,.F.);
#67031=ORIENTED_EDGE('',*,*,#50472,.F.);
#67032=ORIENTED_EDGE('',*,*,#48612,.F.);
#67033=ORIENTED_EDGE('',*,*,#50469,.T.);
#67034=ORIENTED_EDGE('',*,*,#50471,.T.);
#67035=ORIENTED_EDGE('',*,*,#48609,.F.);
#67036=ORIENTED_EDGE('',*,*,#50473,.F.);
#67037=ORIENTED_EDGE('',*,*,#48303,.F.);
#67038=ORIENTED_EDGE('',*,*,#50472,.T.);
#67039=ORIENTED_EDGE('',*,*,#48316,.F.);
#67040=ORIENTED_EDGE('',*,*,#50474,.F.);
#67041=ORIENTED_EDGE('',*,*,#48601,.F.);
#67042=ORIENTED_EDGE('',*,*,#50473,.T.);
#67043=ORIENTED_EDGE('',*,*,#48608,.F.);
#67044=ORIENTED_EDGE('',*,*,#50475,.F.);
#67045=ORIENTED_EDGE('',*,*,#48320,.F.);
#67046=ORIENTED_EDGE('',*,*,#50474,.T.);
#67047=ORIENTED_EDGE('',*,*,#45943,.F.);
#67048=ORIENTED_EDGE('',*,*,#50476,.F.);
#67049=ORIENTED_EDGE('',*,*,#48602,.F.);
#67050=ORIENTED_EDGE('',*,*,#50475,.T.);
#67051=ORIENTED_EDGE('',*,*,#48607,.F.);
#67052=ORIENTED_EDGE('',*,*,#50477,.F.);
#67053=ORIENTED_EDGE('',*,*,#48295,.T.);
#67054=ORIENTED_EDGE('',*,*,#48299,.F.);
#67055=ORIENTED_EDGE('',*,*,#50476,.T.);
#67056=ORIENTED_EDGE('',*,*,#45942,.F.);
#67057=ORIENTED_EDGE('',*,*,#50478,.F.);
#67058=ORIENTED_EDGE('',*,*,#50161,.F.);
#67059=ORIENTED_EDGE('',*,*,#50477,.T.);
#67060=ORIENTED_EDGE('',*,*,#48606,.F.);
#67061=ORIENTED_EDGE('',*,*,#50479,.F.);
#67062=ORIENTED_EDGE('',*,*,#48296,.F.);
#67063=ORIENTED_EDGE('',*,*,#50478,.T.);
#67064=ORIENTED_EDGE('',*,*,#45941,.F.);
#67065=ORIENTED_EDGE('',*,*,#50480,.F.);
#67066=ORIENTED_EDGE('',*,*,#48586,.F.);
#67067=ORIENTED_EDGE('',*,*,#50479,.T.);
#67068=ORIENTED_EDGE('',*,*,#48605,.F.);
#67069=ORIENTED_EDGE('',*,*,#50481,.F.);
#67070=ORIENTED_EDGE('',*,*,#48314,.F.);
#67071=ORIENTED_EDGE('',*,*,#50480,.T.);
#67072=ORIENTED_EDGE('',*,*,#45940,.F.);
#67073=ORIENTED_EDGE('',*,*,#50482,.F.);
#67074=ORIENTED_EDGE('',*,*,#50163,.F.);
#67075=ORIENTED_EDGE('',*,*,#50481,.T.);
#67076=ORIENTED_EDGE('',*,*,#48604,.F.);
#67077=ORIENTED_EDGE('',*,*,#50483,.F.);
#67078=ORIENTED_EDGE('',*,*,#46429,.F.);
#67079=ORIENTED_EDGE('',*,*,#50482,.T.);
#67080=ORIENTED_EDGE('',*,*,#45939,.F.);
#67081=ORIENTED_EDGE('',*,*,#50484,.F.);
#67082=ORIENTED_EDGE('',*,*,#48592,.F.);
#67083=ORIENTED_EDGE('',*,*,#50483,.T.);
#67084=ORIENTED_EDGE('',*,*,#50162,.F.);
#67085=ORIENTED_EDGE('',*,*,#50485,.F.);
#67086=ORIENTED_EDGE('',*,*,#46430,.F.);
#67087=ORIENTED_EDGE('',*,*,#50484,.T.);
#67088=ORIENTED_EDGE('',*,*,#48345,.F.);
#67089=ORIENTED_EDGE('',*,*,#50486,.F.);
#67090=ORIENTED_EDGE('',*,*,#48593,.F.);
#67091=ORIENTED_EDGE('',*,*,#50485,.T.);
#67092=ORIENTED_EDGE('',*,*,#48588,.F.);
#67093=ORIENTED_EDGE('',*,*,#50487,.F.);
#67094=ORIENTED_EDGE('',*,*,#46431,.F.);
#67095=ORIENTED_EDGE('',*,*,#48340,.F.);
#67096=ORIENTED_EDGE('',*,*,#48336,.T.);
#67097=ORIENTED_EDGE('',*,*,#50488,.F.);
#67098=ORIENTED_EDGE('',*,*,#48594,.F.);
#67099=ORIENTED_EDGE('',*,*,#50486,.T.);
#67100=ORIENTED_EDGE('',*,*,#50487,.T.);
#67101=ORIENTED_EDGE('',*,*,#50164,.F.);
#67102=ORIENTED_EDGE('',*,*,#50489,.F.);
#67103=ORIENTED_EDGE('',*,*,#46432,.F.);
#67104=ORIENTED_EDGE('',*,*,#50488,.T.);
#67105=ORIENTED_EDGE('',*,*,#48335,.F.);
#67106=ORIENTED_EDGE('',*,*,#50490,.F.);
#67107=ORIENTED_EDGE('',*,*,#48595,.F.);
#67108=ORIENTED_EDGE('',*,*,#50489,.T.);
#67109=ORIENTED_EDGE('',*,*,#48590,.F.);
#67110=ORIENTED_EDGE('',*,*,#50491,.F.);
#67111=ORIENTED_EDGE('',*,*,#46433,.F.);
#67112=ORIENTED_EDGE('',*,*,#50490,.T.);
#67113=ORIENTED_EDGE('',*,*,#48347,.F.);
#67114=ORIENTED_EDGE('',*,*,#50492,.F.);
#67115=ORIENTED_EDGE('',*,*,#48596,.F.);
#67116=ORIENTED_EDGE('',*,*,#50491,.T.);
#67117=ORIENTED_EDGE('',*,*,#48589,.F.);
#67118=ORIENTED_EDGE('',*,*,#50493,.F.);
#67119=ORIENTED_EDGE('',*,*,#48343,.F.);
#67120=ORIENTED_EDGE('',*,*,#50492,.T.);
#67121=ORIENTED_EDGE('',*,*,#48331,.F.);
#67122=ORIENTED_EDGE('',*,*,#50494,.F.);
#67123=ORIENTED_EDGE('',*,*,#48597,.F.);
#67124=ORIENTED_EDGE('',*,*,#50493,.T.);
#67125=ORIENTED_EDGE('',*,*,#48600,.F.);
#67126=ORIENTED_EDGE('',*,*,#50495,.F.);
#67127=ORIENTED_EDGE('',*,*,#48322,.F.);
#67128=ORIENTED_EDGE('',*,*,#50494,.T.);
#67129=ORIENTED_EDGE('',*,*,#48349,.F.);
#67130=ORIENTED_EDGE('',*,*,#50496,.F.);
#67131=ORIENTED_EDGE('',*,*,#48598,.F.);
#67132=ORIENTED_EDGE('',*,*,#50495,.T.);
#67133=ORIENTED_EDGE('',*,*,#48599,.F.);
#67134=ORIENTED_EDGE('',*,*,#50496,.T.);
#67135=ORIENTED_EDGE('',*,*,#48327,.F.);
#67136=ORIENTED_EDGE('',*,*,#48323,.T.);
#67137=ORIENTED_EDGE('',*,*,#50497,.F.);
#67138=ORIENTED_EDGE('',*,*,#48639,.F.);
#67139=ORIENTED_EDGE('',*,*,#50498,.F.);
#67140=ORIENTED_EDGE('',*,*,#48279,.F.);
#67141=ORIENTED_EDGE('',*,*,#50498,.T.);
#67142=ORIENTED_EDGE('',*,*,#48638,.F.);
#67143=ORIENTED_EDGE('',*,*,#50499,.F.);
#67144=ORIENTED_EDGE('',*,*,#48288,.F.);
#67145=ORIENTED_EDGE('',*,*,#48278,.T.);
#67146=ORIENTED_EDGE('',*,*,#48282,.F.);
#67147=ORIENTED_EDGE('',*,*,#50500,.F.);
#67148=ORIENTED_EDGE('',*,*,#48640,.F.);
#67149=ORIENTED_EDGE('',*,*,#50497,.T.);
#67150=ORIENTED_EDGE('',*,*,#50499,.T.);
#67151=ORIENTED_EDGE('',*,*,#48637,.F.);
#67152=ORIENTED_EDGE('',*,*,#50501,.F.);
#67153=ORIENTED_EDGE('',*,*,#48273,.F.);
#67154=ORIENTED_EDGE('',*,*,#50500,.T.);
#67155=ORIENTED_EDGE('',*,*,#48286,.F.);
#67156=ORIENTED_EDGE('',*,*,#50502,.F.);
#67157=ORIENTED_EDGE('',*,*,#48629,.F.);
#67158=ORIENTED_EDGE('',*,*,#50501,.T.);
#67159=ORIENTED_EDGE('',*,*,#48636,.F.);
#67160=ORIENTED_EDGE('',*,*,#50503,.F.);
#67161=ORIENTED_EDGE('',*,*,#48290,.F.);
#67162=ORIENTED_EDGE('',*,*,#50502,.T.);
#67163=ORIENTED_EDGE('',*,*,#45949,.F.);
#67164=ORIENTED_EDGE('',*,*,#50504,.F.);
#67165=ORIENTED_EDGE('',*,*,#48630,.F.);
#67166=ORIENTED_EDGE('',*,*,#50503,.T.);
#67167=ORIENTED_EDGE('',*,*,#48635,.F.);
#67168=ORIENTED_EDGE('',*,*,#50505,.F.);
#67169=ORIENTED_EDGE('',*,*,#48265,.T.);
#67170=ORIENTED_EDGE('',*,*,#48269,.F.);
#67171=ORIENTED_EDGE('',*,*,#50504,.T.);
#67172=ORIENTED_EDGE('',*,*,#45948,.F.);
#67173=ORIENTED_EDGE('',*,*,#50506,.F.);
#67174=ORIENTED_EDGE('',*,*,#50165,.F.);
#67175=ORIENTED_EDGE('',*,*,#50505,.T.);
#67176=ORIENTED_EDGE('',*,*,#48634,.F.);
#67177=ORIENTED_EDGE('',*,*,#50507,.F.);
#67178=ORIENTED_EDGE('',*,*,#48266,.F.);
#67179=ORIENTED_EDGE('',*,*,#50506,.T.);
#67180=ORIENTED_EDGE('',*,*,#45947,.F.);
#67181=ORIENTED_EDGE('',*,*,#50508,.F.);
#67182=ORIENTED_EDGE('',*,*,#48614,.F.);
#67183=ORIENTED_EDGE('',*,*,#50507,.T.);
#67184=ORIENTED_EDGE('',*,*,#48633,.F.);
#67185=ORIENTED_EDGE('',*,*,#50509,.F.);
#67186=ORIENTED_EDGE('',*,*,#48284,.F.);
#67187=ORIENTED_EDGE('',*,*,#50508,.T.);
#67188=ORIENTED_EDGE('',*,*,#45946,.F.);
#67189=ORIENTED_EDGE('',*,*,#50510,.F.);
#67190=ORIENTED_EDGE('',*,*,#50167,.F.);
#67191=ORIENTED_EDGE('',*,*,#50509,.T.);
#67192=ORIENTED_EDGE('',*,*,#48632,.F.);
#67193=ORIENTED_EDGE('',*,*,#50511,.F.);
#67194=ORIENTED_EDGE('',*,*,#46423,.F.);
#67195=ORIENTED_EDGE('',*,*,#50510,.T.);
#67196=ORIENTED_EDGE('',*,*,#45945,.F.);
#67197=ORIENTED_EDGE('',*,*,#50512,.F.);
#67198=ORIENTED_EDGE('',*,*,#48620,.F.);
#67199=ORIENTED_EDGE('',*,*,#50511,.T.);
#67200=ORIENTED_EDGE('',*,*,#50166,.F.);
#67201=ORIENTED_EDGE('',*,*,#50513,.F.);
#67202=ORIENTED_EDGE('',*,*,#46424,.F.);
#67203=ORIENTED_EDGE('',*,*,#50512,.T.);
#67204=ORIENTED_EDGE('',*,*,#48315,.F.);
#67205=ORIENTED_EDGE('',*,*,#50514,.F.);
#67206=ORIENTED_EDGE('',*,*,#48621,.F.);
#67207=ORIENTED_EDGE('',*,*,#50513,.T.);
#67208=ORIENTED_EDGE('',*,*,#48616,.F.);
#67209=ORIENTED_EDGE('',*,*,#50515,.F.);
#67210=ORIENTED_EDGE('',*,*,#46425,.F.);
#67211=ORIENTED_EDGE('',*,*,#48310,.F.);
#67212=ORIENTED_EDGE('',*,*,#48306,.T.);
#67213=ORIENTED_EDGE('',*,*,#50516,.F.);
#67214=ORIENTED_EDGE('',*,*,#48622,.F.);
#67215=ORIENTED_EDGE('',*,*,#50514,.T.);
#67216=ORIENTED_EDGE('',*,*,#50515,.T.);
#67217=ORIENTED_EDGE('',*,*,#50168,.F.);
#67218=ORIENTED_EDGE('',*,*,#50517,.F.);
#67219=ORIENTED_EDGE('',*,*,#46426,.F.);
#67220=ORIENTED_EDGE('',*,*,#50516,.T.);
#67221=ORIENTED_EDGE('',*,*,#48305,.F.);
#67222=ORIENTED_EDGE('',*,*,#50518,.F.);
#67223=ORIENTED_EDGE('',*,*,#48623,.F.);
#67224=ORIENTED_EDGE('',*,*,#50517,.T.);
#67225=ORIENTED_EDGE('',*,*,#48618,.F.);
#67226=ORIENTED_EDGE('',*,*,#50519,.F.);
#67227=ORIENTED_EDGE('',*,*,#46427,.F.);
#67228=ORIENTED_EDGE('',*,*,#50518,.T.);
#67229=ORIENTED_EDGE('',*,*,#48317,.F.);
#67230=ORIENTED_EDGE('',*,*,#50520,.F.);
#67231=ORIENTED_EDGE('',*,*,#48624,.F.);
#67232=ORIENTED_EDGE('',*,*,#50519,.T.);
#67233=ORIENTED_EDGE('',*,*,#48617,.F.);
#67234=ORIENTED_EDGE('',*,*,#50521,.F.);
#67235=ORIENTED_EDGE('',*,*,#48313,.F.);
#67236=ORIENTED_EDGE('',*,*,#50520,.T.);
#67237=ORIENTED_EDGE('',*,*,#48301,.F.);
#67238=ORIENTED_EDGE('',*,*,#50522,.F.);
#67239=ORIENTED_EDGE('',*,*,#48625,.F.);
#67240=ORIENTED_EDGE('',*,*,#50521,.T.);
#67241=ORIENTED_EDGE('',*,*,#48628,.F.);
#67242=ORIENTED_EDGE('',*,*,#50523,.F.);
#67243=ORIENTED_EDGE('',*,*,#48292,.F.);
#67244=ORIENTED_EDGE('',*,*,#50522,.T.);
#67245=ORIENTED_EDGE('',*,*,#48319,.F.);
#67246=ORIENTED_EDGE('',*,*,#50524,.F.);
#67247=ORIENTED_EDGE('',*,*,#48626,.F.);
#67248=ORIENTED_EDGE('',*,*,#50523,.T.);
#67249=ORIENTED_EDGE('',*,*,#48627,.F.);
#67250=ORIENTED_EDGE('',*,*,#50524,.T.);
#67251=ORIENTED_EDGE('',*,*,#48297,.F.);
#67252=ORIENTED_EDGE('',*,*,#48293,.T.);
#67253=ORIENTED_EDGE('',*,*,#50525,.F.);
#67254=ORIENTED_EDGE('',*,*,#48667,.F.);
#67255=ORIENTED_EDGE('',*,*,#50526,.F.);
#67256=ORIENTED_EDGE('',*,*,#48249,.F.);
#67257=ORIENTED_EDGE('',*,*,#50526,.T.);
#67258=ORIENTED_EDGE('',*,*,#48666,.F.);
#67259=ORIENTED_EDGE('',*,*,#50527,.F.);
#67260=ORIENTED_EDGE('',*,*,#48258,.F.);
#67261=ORIENTED_EDGE('',*,*,#48248,.T.);
#67262=ORIENTED_EDGE('',*,*,#48252,.F.);
#67263=ORIENTED_EDGE('',*,*,#50528,.F.);
#67264=ORIENTED_EDGE('',*,*,#48668,.F.);
#67265=ORIENTED_EDGE('',*,*,#50525,.T.);
#67266=ORIENTED_EDGE('',*,*,#50527,.T.);
#67267=ORIENTED_EDGE('',*,*,#48665,.F.);
#67268=ORIENTED_EDGE('',*,*,#50529,.F.);
#67269=ORIENTED_EDGE('',*,*,#48243,.F.);
#67270=ORIENTED_EDGE('',*,*,#50528,.T.);
#67271=ORIENTED_EDGE('',*,*,#48256,.F.);
#67272=ORIENTED_EDGE('',*,*,#50530,.F.);
#67273=ORIENTED_EDGE('',*,*,#48657,.F.);
#67274=ORIENTED_EDGE('',*,*,#50529,.T.);
#67275=ORIENTED_EDGE('',*,*,#48664,.F.);
#67276=ORIENTED_EDGE('',*,*,#50531,.F.);
#67277=ORIENTED_EDGE('',*,*,#48260,.F.);
#67278=ORIENTED_EDGE('',*,*,#50530,.T.);
#67279=ORIENTED_EDGE('',*,*,#45955,.F.);
#67280=ORIENTED_EDGE('',*,*,#50532,.F.);
#67281=ORIENTED_EDGE('',*,*,#48658,.F.);
#67282=ORIENTED_EDGE('',*,*,#50531,.T.);
#67283=ORIENTED_EDGE('',*,*,#48663,.F.);
#67284=ORIENTED_EDGE('',*,*,#50533,.F.);
#67285=ORIENTED_EDGE('',*,*,#48235,.T.);
#67286=ORIENTED_EDGE('',*,*,#48239,.F.);
#67287=ORIENTED_EDGE('',*,*,#50532,.T.);
#67288=ORIENTED_EDGE('',*,*,#45954,.F.);
#67289=ORIENTED_EDGE('',*,*,#50534,.F.);
#67290=ORIENTED_EDGE('',*,*,#50169,.F.);
#67291=ORIENTED_EDGE('',*,*,#50533,.T.);
#67292=ORIENTED_EDGE('',*,*,#48662,.F.);
#67293=ORIENTED_EDGE('',*,*,#50535,.F.);
#67294=ORIENTED_EDGE('',*,*,#48236,.F.);
#67295=ORIENTED_EDGE('',*,*,#50534,.T.);
#67296=ORIENTED_EDGE('',*,*,#45953,.F.);
#67297=ORIENTED_EDGE('',*,*,#50536,.F.);
#67298=ORIENTED_EDGE('',*,*,#48642,.F.);
#67299=ORIENTED_EDGE('',*,*,#50535,.T.);
#67300=ORIENTED_EDGE('',*,*,#48661,.F.);
#67301=ORIENTED_EDGE('',*,*,#50537,.F.);
#67302=ORIENTED_EDGE('',*,*,#48254,.F.);
#67303=ORIENTED_EDGE('',*,*,#50536,.T.);
#67304=ORIENTED_EDGE('',*,*,#45952,.F.);
#67305=ORIENTED_EDGE('',*,*,#50538,.F.);
#67306=ORIENTED_EDGE('',*,*,#50171,.F.);
#67307=ORIENTED_EDGE('',*,*,#50537,.T.);
#67308=ORIENTED_EDGE('',*,*,#48660,.F.);
#67309=ORIENTED_EDGE('',*,*,#50539,.F.);
#67310=ORIENTED_EDGE('',*,*,#46417,.F.);
#67311=ORIENTED_EDGE('',*,*,#50538,.T.);
#67312=ORIENTED_EDGE('',*,*,#45951,.F.);
#67313=ORIENTED_EDGE('',*,*,#50540,.F.);
#67314=ORIENTED_EDGE('',*,*,#48648,.F.);
#67315=ORIENTED_EDGE('',*,*,#50539,.T.);
#67316=ORIENTED_EDGE('',*,*,#50170,.F.);
#67317=ORIENTED_EDGE('',*,*,#50541,.F.);
#67318=ORIENTED_EDGE('',*,*,#46418,.F.);
#67319=ORIENTED_EDGE('',*,*,#50540,.T.);
#67320=ORIENTED_EDGE('',*,*,#48285,.F.);
#67321=ORIENTED_EDGE('',*,*,#50542,.F.);
#67322=ORIENTED_EDGE('',*,*,#48649,.F.);
#67323=ORIENTED_EDGE('',*,*,#50541,.T.);
#67324=ORIENTED_EDGE('',*,*,#48644,.F.);
#67325=ORIENTED_EDGE('',*,*,#50543,.F.);
#67326=ORIENTED_EDGE('',*,*,#46419,.F.);
#67327=ORIENTED_EDGE('',*,*,#48280,.F.);
#67328=ORIENTED_EDGE('',*,*,#48276,.T.);
#67329=ORIENTED_EDGE('',*,*,#50544,.F.);
#67330=ORIENTED_EDGE('',*,*,#48650,.F.);
#67331=ORIENTED_EDGE('',*,*,#50542,.T.);
#67332=ORIENTED_EDGE('',*,*,#50543,.T.);
#67333=ORIENTED_EDGE('',*,*,#50172,.F.);
#67334=ORIENTED_EDGE('',*,*,#50545,.F.);
#67335=ORIENTED_EDGE('',*,*,#46420,.F.);
#67336=ORIENTED_EDGE('',*,*,#50544,.T.);
#67337=ORIENTED_EDGE('',*,*,#48275,.F.);
#67338=ORIENTED_EDGE('',*,*,#50546,.F.);
#67339=ORIENTED_EDGE('',*,*,#48651,.F.);
#67340=ORIENTED_EDGE('',*,*,#50545,.T.);
#67341=ORIENTED_EDGE('',*,*,#48646,.F.);
#67342=ORIENTED_EDGE('',*,*,#50547,.F.);
#67343=ORIENTED_EDGE('',*,*,#46421,.F.);
#67344=ORIENTED_EDGE('',*,*,#50546,.T.);
#67345=ORIENTED_EDGE('',*,*,#48287,.F.);
#67346=ORIENTED_EDGE('',*,*,#50548,.F.);
#67347=ORIENTED_EDGE('',*,*,#48652,.F.);
#67348=ORIENTED_EDGE('',*,*,#50547,.T.);
#67349=ORIENTED_EDGE('',*,*,#48645,.F.);
#67350=ORIENTED_EDGE('',*,*,#50549,.F.);
#67351=ORIENTED_EDGE('',*,*,#48283,.F.);
#67352=ORIENTED_EDGE('',*,*,#50548,.T.);
#67353=ORIENTED_EDGE('',*,*,#48271,.F.);
#67354=ORIENTED_EDGE('',*,*,#50550,.F.);
#67355=ORIENTED_EDGE('',*,*,#48653,.F.);
#67356=ORIENTED_EDGE('',*,*,#50549,.T.);
#67357=ORIENTED_EDGE('',*,*,#48656,.F.);
#67358=ORIENTED_EDGE('',*,*,#50551,.F.);
#67359=ORIENTED_EDGE('',*,*,#48262,.F.);
#67360=ORIENTED_EDGE('',*,*,#50550,.T.);
#67361=ORIENTED_EDGE('',*,*,#48289,.F.);
#67362=ORIENTED_EDGE('',*,*,#50552,.F.);
#67363=ORIENTED_EDGE('',*,*,#48654,.F.);
#67364=ORIENTED_EDGE('',*,*,#50551,.T.);
#67365=ORIENTED_EDGE('',*,*,#48655,.F.);
#67366=ORIENTED_EDGE('',*,*,#50552,.T.);
#67367=ORIENTED_EDGE('',*,*,#48267,.F.);
#67368=ORIENTED_EDGE('',*,*,#48263,.T.);
#67369=ORIENTED_EDGE('',*,*,#50553,.F.);
#67370=ORIENTED_EDGE('',*,*,#48695,.F.);
#67371=ORIENTED_EDGE('',*,*,#50554,.F.);
#67372=ORIENTED_EDGE('',*,*,#48219,.F.);
#67373=ORIENTED_EDGE('',*,*,#50554,.T.);
#67374=ORIENTED_EDGE('',*,*,#48694,.F.);
#67375=ORIENTED_EDGE('',*,*,#50555,.F.);
#67376=ORIENTED_EDGE('',*,*,#48228,.F.);
#67377=ORIENTED_EDGE('',*,*,#48218,.T.);
#67378=ORIENTED_EDGE('',*,*,#48222,.F.);
#67379=ORIENTED_EDGE('',*,*,#50556,.F.);
#67380=ORIENTED_EDGE('',*,*,#48696,.F.);
#67381=ORIENTED_EDGE('',*,*,#50553,.T.);
#67382=ORIENTED_EDGE('',*,*,#50555,.T.);
#67383=ORIENTED_EDGE('',*,*,#48693,.F.);
#67384=ORIENTED_EDGE('',*,*,#50557,.F.);
#67385=ORIENTED_EDGE('',*,*,#48213,.F.);
#67386=ORIENTED_EDGE('',*,*,#50556,.T.);
#67387=ORIENTED_EDGE('',*,*,#48226,.F.);
#67388=ORIENTED_EDGE('',*,*,#50558,.F.);
#67389=ORIENTED_EDGE('',*,*,#48685,.F.);
#67390=ORIENTED_EDGE('',*,*,#50557,.T.);
#67391=ORIENTED_EDGE('',*,*,#48692,.F.);
#67392=ORIENTED_EDGE('',*,*,#50559,.F.);
#67393=ORIENTED_EDGE('',*,*,#48230,.F.);
#67394=ORIENTED_EDGE('',*,*,#50558,.T.);
#67395=ORIENTED_EDGE('',*,*,#45961,.F.);
#67396=ORIENTED_EDGE('',*,*,#50560,.F.);
#67397=ORIENTED_EDGE('',*,*,#48686,.F.);
#67398=ORIENTED_EDGE('',*,*,#50559,.T.);
#67399=ORIENTED_EDGE('',*,*,#48691,.F.);
#67400=ORIENTED_EDGE('',*,*,#50561,.F.);
#67401=ORIENTED_EDGE('',*,*,#48205,.T.);
#67402=ORIENTED_EDGE('',*,*,#48209,.F.);
#67403=ORIENTED_EDGE('',*,*,#50560,.T.);
#67404=ORIENTED_EDGE('',*,*,#45960,.F.);
#67405=ORIENTED_EDGE('',*,*,#50562,.F.);
#67406=ORIENTED_EDGE('',*,*,#50173,.F.);
#67407=ORIENTED_EDGE('',*,*,#50561,.T.);
#67408=ORIENTED_EDGE('',*,*,#48690,.F.);
#67409=ORIENTED_EDGE('',*,*,#50563,.F.);
#67410=ORIENTED_EDGE('',*,*,#48206,.F.);
#67411=ORIENTED_EDGE('',*,*,#50562,.T.);
#67412=ORIENTED_EDGE('',*,*,#45959,.F.);
#67413=ORIENTED_EDGE('',*,*,#50564,.F.);
#67414=ORIENTED_EDGE('',*,*,#48670,.F.);
#67415=ORIENTED_EDGE('',*,*,#50563,.T.);
#67416=ORIENTED_EDGE('',*,*,#48689,.F.);
#67417=ORIENTED_EDGE('',*,*,#50565,.F.);
#67418=ORIENTED_EDGE('',*,*,#48224,.F.);
#67419=ORIENTED_EDGE('',*,*,#50564,.T.);
#67420=ORIENTED_EDGE('',*,*,#45958,.F.);
#67421=ORIENTED_EDGE('',*,*,#50566,.F.);
#67422=ORIENTED_EDGE('',*,*,#50175,.F.);
#67423=ORIENTED_EDGE('',*,*,#50565,.T.);
#67424=ORIENTED_EDGE('',*,*,#48688,.F.);
#67425=ORIENTED_EDGE('',*,*,#50567,.F.);
#67426=ORIENTED_EDGE('',*,*,#46411,.F.);
#67427=ORIENTED_EDGE('',*,*,#50566,.T.);
#67428=ORIENTED_EDGE('',*,*,#45957,.F.);
#67429=ORIENTED_EDGE('',*,*,#50568,.F.);
#67430=ORIENTED_EDGE('',*,*,#48676,.F.);
#67431=ORIENTED_EDGE('',*,*,#50567,.T.);
#67432=ORIENTED_EDGE('',*,*,#50174,.F.);
#67433=ORIENTED_EDGE('',*,*,#50569,.F.);
#67434=ORIENTED_EDGE('',*,*,#46412,.F.);
#67435=ORIENTED_EDGE('',*,*,#50568,.T.);
#67436=ORIENTED_EDGE('',*,*,#48255,.F.);
#67437=ORIENTED_EDGE('',*,*,#50570,.F.);
#67438=ORIENTED_EDGE('',*,*,#48677,.F.);
#67439=ORIENTED_EDGE('',*,*,#50569,.T.);
#67440=ORIENTED_EDGE('',*,*,#48672,.F.);
#67441=ORIENTED_EDGE('',*,*,#50571,.F.);
#67442=ORIENTED_EDGE('',*,*,#46413,.F.);
#67443=ORIENTED_EDGE('',*,*,#48250,.F.);
#67444=ORIENTED_EDGE('',*,*,#48246,.T.);
#67445=ORIENTED_EDGE('',*,*,#50572,.F.);
#67446=ORIENTED_EDGE('',*,*,#48678,.F.);
#67447=ORIENTED_EDGE('',*,*,#50570,.T.);
#67448=ORIENTED_EDGE('',*,*,#50571,.T.);
#67449=ORIENTED_EDGE('',*,*,#50176,.F.);
#67450=ORIENTED_EDGE('',*,*,#50573,.F.);
#67451=ORIENTED_EDGE('',*,*,#46414,.F.);
#67452=ORIENTED_EDGE('',*,*,#50572,.T.);
#67453=ORIENTED_EDGE('',*,*,#48245,.F.);
#67454=ORIENTED_EDGE('',*,*,#50574,.F.);
#67455=ORIENTED_EDGE('',*,*,#48679,.F.);
#67456=ORIENTED_EDGE('',*,*,#50573,.T.);
#67457=ORIENTED_EDGE('',*,*,#48674,.F.);
#67458=ORIENTED_EDGE('',*,*,#50575,.F.);
#67459=ORIENTED_EDGE('',*,*,#46415,.F.);
#67460=ORIENTED_EDGE('',*,*,#50574,.T.);
#67461=ORIENTED_EDGE('',*,*,#48257,.F.);
#67462=ORIENTED_EDGE('',*,*,#50576,.F.);
#67463=ORIENTED_EDGE('',*,*,#48680,.F.);
#67464=ORIENTED_EDGE('',*,*,#50575,.T.);
#67465=ORIENTED_EDGE('',*,*,#48673,.F.);
#67466=ORIENTED_EDGE('',*,*,#50577,.F.);
#67467=ORIENTED_EDGE('',*,*,#48253,.F.);
#67468=ORIENTED_EDGE('',*,*,#50576,.T.);
#67469=ORIENTED_EDGE('',*,*,#48241,.F.);
#67470=ORIENTED_EDGE('',*,*,#50578,.F.);
#67471=ORIENTED_EDGE('',*,*,#48681,.F.);
#67472=ORIENTED_EDGE('',*,*,#50577,.T.);
#67473=ORIENTED_EDGE('',*,*,#48684,.F.);
#67474=ORIENTED_EDGE('',*,*,#50579,.F.);
#67475=ORIENTED_EDGE('',*,*,#48232,.F.);
#67476=ORIENTED_EDGE('',*,*,#50578,.T.);
#67477=ORIENTED_EDGE('',*,*,#48259,.F.);
#67478=ORIENTED_EDGE('',*,*,#50580,.F.);
#67479=ORIENTED_EDGE('',*,*,#48682,.F.);
#67480=ORIENTED_EDGE('',*,*,#50579,.T.);
#67481=ORIENTED_EDGE('',*,*,#48683,.F.);
#67482=ORIENTED_EDGE('',*,*,#50580,.T.);
#67483=ORIENTED_EDGE('',*,*,#48237,.F.);
#67484=ORIENTED_EDGE('',*,*,#48233,.T.);
#67485=ORIENTED_EDGE('',*,*,#50581,.F.);
#67486=ORIENTED_EDGE('',*,*,#48723,.F.);
#67487=ORIENTED_EDGE('',*,*,#50582,.F.);
#67488=ORIENTED_EDGE('',*,*,#48189,.F.);
#67489=ORIENTED_EDGE('',*,*,#50582,.T.);
#67490=ORIENTED_EDGE('',*,*,#48722,.F.);
#67491=ORIENTED_EDGE('',*,*,#50583,.F.);
#67492=ORIENTED_EDGE('',*,*,#48198,.F.);
#67493=ORIENTED_EDGE('',*,*,#48188,.T.);
#67494=ORIENTED_EDGE('',*,*,#48192,.F.);
#67495=ORIENTED_EDGE('',*,*,#50584,.F.);
#67496=ORIENTED_EDGE('',*,*,#48724,.F.);
#67497=ORIENTED_EDGE('',*,*,#50581,.T.);
#67498=ORIENTED_EDGE('',*,*,#50583,.T.);
#67499=ORIENTED_EDGE('',*,*,#48721,.F.);
#67500=ORIENTED_EDGE('',*,*,#50585,.F.);
#67501=ORIENTED_EDGE('',*,*,#48183,.F.);
#67502=ORIENTED_EDGE('',*,*,#50584,.T.);
#67503=ORIENTED_EDGE('',*,*,#48196,.F.);
#67504=ORIENTED_EDGE('',*,*,#50586,.F.);
#67505=ORIENTED_EDGE('',*,*,#48713,.F.);
#67506=ORIENTED_EDGE('',*,*,#50585,.T.);
#67507=ORIENTED_EDGE('',*,*,#48720,.F.);
#67508=ORIENTED_EDGE('',*,*,#50587,.F.);
#67509=ORIENTED_EDGE('',*,*,#48200,.F.);
#67510=ORIENTED_EDGE('',*,*,#50586,.T.);
#67511=ORIENTED_EDGE('',*,*,#45967,.F.);
#67512=ORIENTED_EDGE('',*,*,#50588,.F.);
#67513=ORIENTED_EDGE('',*,*,#48714,.F.);
#67514=ORIENTED_EDGE('',*,*,#50587,.T.);
#67515=ORIENTED_EDGE('',*,*,#48719,.F.);
#67516=ORIENTED_EDGE('',*,*,#50589,.F.);
#67517=ORIENTED_EDGE('',*,*,#48175,.T.);
#67518=ORIENTED_EDGE('',*,*,#48179,.F.);
#67519=ORIENTED_EDGE('',*,*,#50588,.T.);
#67520=ORIENTED_EDGE('',*,*,#45966,.F.);
#67521=ORIENTED_EDGE('',*,*,#50590,.F.);
#67522=ORIENTED_EDGE('',*,*,#50177,.F.);
#67523=ORIENTED_EDGE('',*,*,#50589,.T.);
#67524=ORIENTED_EDGE('',*,*,#48718,.F.);
#67525=ORIENTED_EDGE('',*,*,#50591,.F.);
#67526=ORIENTED_EDGE('',*,*,#48176,.F.);
#67527=ORIENTED_EDGE('',*,*,#50590,.T.);
#67528=ORIENTED_EDGE('',*,*,#45965,.F.);
#67529=ORIENTED_EDGE('',*,*,#50592,.F.);
#67530=ORIENTED_EDGE('',*,*,#48698,.F.);
#67531=ORIENTED_EDGE('',*,*,#50591,.T.);
#67532=ORIENTED_EDGE('',*,*,#48717,.F.);
#67533=ORIENTED_EDGE('',*,*,#50593,.F.);
#67534=ORIENTED_EDGE('',*,*,#48194,.F.);
#67535=ORIENTED_EDGE('',*,*,#50592,.T.);
#67536=ORIENTED_EDGE('',*,*,#45964,.F.);
#67537=ORIENTED_EDGE('',*,*,#50594,.F.);
#67538=ORIENTED_EDGE('',*,*,#50179,.F.);
#67539=ORIENTED_EDGE('',*,*,#50593,.T.);
#67540=ORIENTED_EDGE('',*,*,#48716,.F.);
#67541=ORIENTED_EDGE('',*,*,#50595,.F.);
#67542=ORIENTED_EDGE('',*,*,#46405,.F.);
#67543=ORIENTED_EDGE('',*,*,#50594,.T.);
#67544=ORIENTED_EDGE('',*,*,#45963,.F.);
#67545=ORIENTED_EDGE('',*,*,#50596,.F.);
#67546=ORIENTED_EDGE('',*,*,#48704,.F.);
#67547=ORIENTED_EDGE('',*,*,#50595,.T.);
#67548=ORIENTED_EDGE('',*,*,#50178,.F.);
#67549=ORIENTED_EDGE('',*,*,#50597,.F.);
#67550=ORIENTED_EDGE('',*,*,#46406,.F.);
#67551=ORIENTED_EDGE('',*,*,#50596,.T.);
#67552=ORIENTED_EDGE('',*,*,#48225,.F.);
#67553=ORIENTED_EDGE('',*,*,#50598,.F.);
#67554=ORIENTED_EDGE('',*,*,#48705,.F.);
#67555=ORIENTED_EDGE('',*,*,#50597,.T.);
#67556=ORIENTED_EDGE('',*,*,#48700,.F.);
#67557=ORIENTED_EDGE('',*,*,#50599,.F.);
#67558=ORIENTED_EDGE('',*,*,#46407,.F.);
#67559=ORIENTED_EDGE('',*,*,#48220,.F.);
#67560=ORIENTED_EDGE('',*,*,#48216,.T.);
#67561=ORIENTED_EDGE('',*,*,#50600,.F.);
#67562=ORIENTED_EDGE('',*,*,#48706,.F.);
#67563=ORIENTED_EDGE('',*,*,#50598,.T.);
#67564=ORIENTED_EDGE('',*,*,#50599,.T.);
#67565=ORIENTED_EDGE('',*,*,#50180,.F.);
#67566=ORIENTED_EDGE('',*,*,#50601,.F.);
#67567=ORIENTED_EDGE('',*,*,#46408,.F.);
#67568=ORIENTED_EDGE('',*,*,#50600,.T.);
#67569=ORIENTED_EDGE('',*,*,#48215,.F.);
#67570=ORIENTED_EDGE('',*,*,#50602,.F.);
#67571=ORIENTED_EDGE('',*,*,#48707,.F.);
#67572=ORIENTED_EDGE('',*,*,#50601,.T.);
#67573=ORIENTED_EDGE('',*,*,#48702,.F.);
#67574=ORIENTED_EDGE('',*,*,#50603,.F.);
#67575=ORIENTED_EDGE('',*,*,#46409,.F.);
#67576=ORIENTED_EDGE('',*,*,#50602,.T.);
#67577=ORIENTED_EDGE('',*,*,#48227,.F.);
#67578=ORIENTED_EDGE('',*,*,#50604,.F.);
#67579=ORIENTED_EDGE('',*,*,#48708,.F.);
#67580=ORIENTED_EDGE('',*,*,#50603,.T.);
#67581=ORIENTED_EDGE('',*,*,#48701,.F.);
#67582=ORIENTED_EDGE('',*,*,#50605,.F.);
#67583=ORIENTED_EDGE('',*,*,#48223,.F.);
#67584=ORIENTED_EDGE('',*,*,#50604,.T.);
#67585=ORIENTED_EDGE('',*,*,#48211,.F.);
#67586=ORIENTED_EDGE('',*,*,#50606,.F.);
#67587=ORIENTED_EDGE('',*,*,#48709,.F.);
#67588=ORIENTED_EDGE('',*,*,#50605,.T.);
#67589=ORIENTED_EDGE('',*,*,#48712,.F.);
#67590=ORIENTED_EDGE('',*,*,#50607,.F.);
#67591=ORIENTED_EDGE('',*,*,#48202,.F.);
#67592=ORIENTED_EDGE('',*,*,#50606,.T.);
#67593=ORIENTED_EDGE('',*,*,#48229,.F.);
#67594=ORIENTED_EDGE('',*,*,#50608,.F.);
#67595=ORIENTED_EDGE('',*,*,#48710,.F.);
#67596=ORIENTED_EDGE('',*,*,#50607,.T.);
#67597=ORIENTED_EDGE('',*,*,#48711,.F.);
#67598=ORIENTED_EDGE('',*,*,#50608,.T.);
#67599=ORIENTED_EDGE('',*,*,#48207,.F.);
#67600=ORIENTED_EDGE('',*,*,#48203,.T.);
#67601=ORIENTED_EDGE('',*,*,#50609,.F.);
#67602=ORIENTED_EDGE('',*,*,#48751,.F.);
#67603=ORIENTED_EDGE('',*,*,#50610,.F.);
#67604=ORIENTED_EDGE('',*,*,#48159,.F.);
#67605=ORIENTED_EDGE('',*,*,#50610,.T.);
#67606=ORIENTED_EDGE('',*,*,#48750,.F.);
#67607=ORIENTED_EDGE('',*,*,#50611,.F.);
#67608=ORIENTED_EDGE('',*,*,#48168,.F.);
#67609=ORIENTED_EDGE('',*,*,#48158,.T.);
#67610=ORIENTED_EDGE('',*,*,#48162,.F.);
#67611=ORIENTED_EDGE('',*,*,#50612,.F.);
#67612=ORIENTED_EDGE('',*,*,#48752,.F.);
#67613=ORIENTED_EDGE('',*,*,#50609,.T.);
#67614=ORIENTED_EDGE('',*,*,#50611,.T.);
#67615=ORIENTED_EDGE('',*,*,#48749,.F.);
#67616=ORIENTED_EDGE('',*,*,#50613,.F.);
#67617=ORIENTED_EDGE('',*,*,#48153,.F.);
#67618=ORIENTED_EDGE('',*,*,#50612,.T.);
#67619=ORIENTED_EDGE('',*,*,#48166,.F.);
#67620=ORIENTED_EDGE('',*,*,#50614,.F.);
#67621=ORIENTED_EDGE('',*,*,#48741,.F.);
#67622=ORIENTED_EDGE('',*,*,#50613,.T.);
#67623=ORIENTED_EDGE('',*,*,#48748,.F.);
#67624=ORIENTED_EDGE('',*,*,#50615,.F.);
#67625=ORIENTED_EDGE('',*,*,#48170,.F.);
#67626=ORIENTED_EDGE('',*,*,#50614,.T.);
#67627=ORIENTED_EDGE('',*,*,#45973,.F.);
#67628=ORIENTED_EDGE('',*,*,#50616,.F.);
#67629=ORIENTED_EDGE('',*,*,#48742,.F.);
#67630=ORIENTED_EDGE('',*,*,#50615,.T.);
#67631=ORIENTED_EDGE('',*,*,#48747,.F.);
#67632=ORIENTED_EDGE('',*,*,#50617,.F.);
#67633=ORIENTED_EDGE('',*,*,#48145,.T.);
#67634=ORIENTED_EDGE('',*,*,#48149,.F.);
#67635=ORIENTED_EDGE('',*,*,#50616,.T.);
#67636=ORIENTED_EDGE('',*,*,#45972,.F.);
#67637=ORIENTED_EDGE('',*,*,#50618,.F.);
#67638=ORIENTED_EDGE('',*,*,#50181,.F.);
#67639=ORIENTED_EDGE('',*,*,#50617,.T.);
#67640=ORIENTED_EDGE('',*,*,#48746,.F.);
#67641=ORIENTED_EDGE('',*,*,#50619,.F.);
#67642=ORIENTED_EDGE('',*,*,#48146,.F.);
#67643=ORIENTED_EDGE('',*,*,#50618,.T.);
#67644=ORIENTED_EDGE('',*,*,#45971,.F.);
#67645=ORIENTED_EDGE('',*,*,#50620,.F.);
#67646=ORIENTED_EDGE('',*,*,#48726,.F.);
#67647=ORIENTED_EDGE('',*,*,#50619,.T.);
#67648=ORIENTED_EDGE('',*,*,#48745,.F.);
#67649=ORIENTED_EDGE('',*,*,#50621,.F.);
#67650=ORIENTED_EDGE('',*,*,#48164,.F.);
#67651=ORIENTED_EDGE('',*,*,#50620,.T.);
#67652=ORIENTED_EDGE('',*,*,#45970,.F.);
#67653=ORIENTED_EDGE('',*,*,#50622,.F.);
#67654=ORIENTED_EDGE('',*,*,#50183,.F.);
#67655=ORIENTED_EDGE('',*,*,#50621,.T.);
#67656=ORIENTED_EDGE('',*,*,#48744,.F.);
#67657=ORIENTED_EDGE('',*,*,#50623,.F.);
#67658=ORIENTED_EDGE('',*,*,#46399,.F.);
#67659=ORIENTED_EDGE('',*,*,#50622,.T.);
#67660=ORIENTED_EDGE('',*,*,#45969,.F.);
#67661=ORIENTED_EDGE('',*,*,#50624,.F.);
#67662=ORIENTED_EDGE('',*,*,#48732,.F.);
#67663=ORIENTED_EDGE('',*,*,#50623,.T.);
#67664=ORIENTED_EDGE('',*,*,#50182,.F.);
#67665=ORIENTED_EDGE('',*,*,#50625,.F.);
#67666=ORIENTED_EDGE('',*,*,#46400,.F.);
#67667=ORIENTED_EDGE('',*,*,#50624,.T.);
#67668=ORIENTED_EDGE('',*,*,#48195,.F.);
#67669=ORIENTED_EDGE('',*,*,#50626,.F.);
#67670=ORIENTED_EDGE('',*,*,#48733,.F.);
#67671=ORIENTED_EDGE('',*,*,#50625,.T.);
#67672=ORIENTED_EDGE('',*,*,#48728,.F.);
#67673=ORIENTED_EDGE('',*,*,#50627,.F.);
#67674=ORIENTED_EDGE('',*,*,#46401,.F.);
#67675=ORIENTED_EDGE('',*,*,#48190,.F.);
#67676=ORIENTED_EDGE('',*,*,#48186,.T.);
#67677=ORIENTED_EDGE('',*,*,#50628,.F.);
#67678=ORIENTED_EDGE('',*,*,#48734,.F.);
#67679=ORIENTED_EDGE('',*,*,#50626,.T.);
#67680=ORIENTED_EDGE('',*,*,#50627,.T.);
#67681=ORIENTED_EDGE('',*,*,#50184,.F.);
#67682=ORIENTED_EDGE('',*,*,#50629,.F.);
#67683=ORIENTED_EDGE('',*,*,#46402,.F.);
#67684=ORIENTED_EDGE('',*,*,#50628,.T.);
#67685=ORIENTED_EDGE('',*,*,#48185,.F.);
#67686=ORIENTED_EDGE('',*,*,#50630,.F.);
#67687=ORIENTED_EDGE('',*,*,#48735,.F.);
#67688=ORIENTED_EDGE('',*,*,#50629,.T.);
#67689=ORIENTED_EDGE('',*,*,#48730,.F.);
#67690=ORIENTED_EDGE('',*,*,#50631,.F.);
#67691=ORIENTED_EDGE('',*,*,#46403,.F.);
#67692=ORIENTED_EDGE('',*,*,#50630,.T.);
#67693=ORIENTED_EDGE('',*,*,#48197,.F.);
#67694=ORIENTED_EDGE('',*,*,#50632,.F.);
#67695=ORIENTED_EDGE('',*,*,#48736,.F.);
#67696=ORIENTED_EDGE('',*,*,#50631,.T.);
#67697=ORIENTED_EDGE('',*,*,#48729,.F.);
#67698=ORIENTED_EDGE('',*,*,#50633,.F.);
#67699=ORIENTED_EDGE('',*,*,#48193,.F.);
#67700=ORIENTED_EDGE('',*,*,#50632,.T.);
#67701=ORIENTED_EDGE('',*,*,#48181,.F.);
#67702=ORIENTED_EDGE('',*,*,#50634,.F.);
#67703=ORIENTED_EDGE('',*,*,#48737,.F.);
#67704=ORIENTED_EDGE('',*,*,#50633,.T.);
#67705=ORIENTED_EDGE('',*,*,#48740,.F.);
#67706=ORIENTED_EDGE('',*,*,#50635,.F.);
#67707=ORIENTED_EDGE('',*,*,#48172,.F.);
#67708=ORIENTED_EDGE('',*,*,#50634,.T.);
#67709=ORIENTED_EDGE('',*,*,#48199,.F.);
#67710=ORIENTED_EDGE('',*,*,#50636,.F.);
#67711=ORIENTED_EDGE('',*,*,#48738,.F.);
#67712=ORIENTED_EDGE('',*,*,#50635,.T.);
#67713=ORIENTED_EDGE('',*,*,#48739,.F.);
#67714=ORIENTED_EDGE('',*,*,#50636,.T.);
#67715=ORIENTED_EDGE('',*,*,#48177,.F.);
#67716=ORIENTED_EDGE('',*,*,#48173,.T.);
#67717=ORIENTED_EDGE('',*,*,#50637,.F.);
#67718=ORIENTED_EDGE('',*,*,#48779,.F.);
#67719=ORIENTED_EDGE('',*,*,#50638,.F.);
#67720=ORIENTED_EDGE('',*,*,#48129,.F.);
#67721=ORIENTED_EDGE('',*,*,#50638,.T.);
#67722=ORIENTED_EDGE('',*,*,#48778,.F.);
#67723=ORIENTED_EDGE('',*,*,#50639,.F.);
#67724=ORIENTED_EDGE('',*,*,#48138,.F.);
#67725=ORIENTED_EDGE('',*,*,#48128,.T.);
#67726=ORIENTED_EDGE('',*,*,#48132,.F.);
#67727=ORIENTED_EDGE('',*,*,#50640,.F.);
#67728=ORIENTED_EDGE('',*,*,#48780,.F.);
#67729=ORIENTED_EDGE('',*,*,#50637,.T.);
#67730=ORIENTED_EDGE('',*,*,#50639,.T.);
#67731=ORIENTED_EDGE('',*,*,#48777,.F.);
#67732=ORIENTED_EDGE('',*,*,#50641,.F.);
#67733=ORIENTED_EDGE('',*,*,#48123,.F.);
#67734=ORIENTED_EDGE('',*,*,#50640,.T.);
#67735=ORIENTED_EDGE('',*,*,#48136,.F.);
#67736=ORIENTED_EDGE('',*,*,#50642,.F.);
#67737=ORIENTED_EDGE('',*,*,#48769,.F.);
#67738=ORIENTED_EDGE('',*,*,#50641,.T.);
#67739=ORIENTED_EDGE('',*,*,#48776,.F.);
#67740=ORIENTED_EDGE('',*,*,#50643,.F.);
#67741=ORIENTED_EDGE('',*,*,#48140,.F.);
#67742=ORIENTED_EDGE('',*,*,#50642,.T.);
#67743=ORIENTED_EDGE('',*,*,#45979,.F.);
#67744=ORIENTED_EDGE('',*,*,#50644,.F.);
#67745=ORIENTED_EDGE('',*,*,#48770,.F.);
#67746=ORIENTED_EDGE('',*,*,#50643,.T.);
#67747=ORIENTED_EDGE('',*,*,#48775,.F.);
#67748=ORIENTED_EDGE('',*,*,#50645,.F.);
#67749=ORIENTED_EDGE('',*,*,#48115,.T.);
#67750=ORIENTED_EDGE('',*,*,#48119,.F.);
#67751=ORIENTED_EDGE('',*,*,#50644,.T.);
#67752=ORIENTED_EDGE('',*,*,#45978,.F.);
#67753=ORIENTED_EDGE('',*,*,#50646,.F.);
#67754=ORIENTED_EDGE('',*,*,#50185,.F.);
#67755=ORIENTED_EDGE('',*,*,#50645,.T.);
#67756=ORIENTED_EDGE('',*,*,#48774,.F.);
#67757=ORIENTED_EDGE('',*,*,#50647,.F.);
#67758=ORIENTED_EDGE('',*,*,#48116,.F.);
#67759=ORIENTED_EDGE('',*,*,#50646,.T.);
#67760=ORIENTED_EDGE('',*,*,#45977,.F.);
#67761=ORIENTED_EDGE('',*,*,#50648,.F.);
#67762=ORIENTED_EDGE('',*,*,#48754,.F.);
#67763=ORIENTED_EDGE('',*,*,#50647,.T.);
#67764=ORIENTED_EDGE('',*,*,#48773,.F.);
#67765=ORIENTED_EDGE('',*,*,#50649,.F.);
#67766=ORIENTED_EDGE('',*,*,#48134,.F.);
#67767=ORIENTED_EDGE('',*,*,#50648,.T.);
#67768=ORIENTED_EDGE('',*,*,#45976,.F.);
#67769=ORIENTED_EDGE('',*,*,#50650,.F.);
#67770=ORIENTED_EDGE('',*,*,#50187,.F.);
#67771=ORIENTED_EDGE('',*,*,#50649,.T.);
#67772=ORIENTED_EDGE('',*,*,#48772,.F.);
#67773=ORIENTED_EDGE('',*,*,#50651,.F.);
#67774=ORIENTED_EDGE('',*,*,#46393,.F.);
#67775=ORIENTED_EDGE('',*,*,#50650,.T.);
#67776=ORIENTED_EDGE('',*,*,#45975,.F.);
#67777=ORIENTED_EDGE('',*,*,#50652,.F.);
#67778=ORIENTED_EDGE('',*,*,#48760,.F.);
#67779=ORIENTED_EDGE('',*,*,#50651,.T.);
#67780=ORIENTED_EDGE('',*,*,#50186,.F.);
#67781=ORIENTED_EDGE('',*,*,#50653,.F.);
#67782=ORIENTED_EDGE('',*,*,#46394,.F.);
#67783=ORIENTED_EDGE('',*,*,#50652,.T.);
#67784=ORIENTED_EDGE('',*,*,#48165,.F.);
#67785=ORIENTED_EDGE('',*,*,#50654,.F.);
#67786=ORIENTED_EDGE('',*,*,#48761,.F.);
#67787=ORIENTED_EDGE('',*,*,#50653,.T.);
#67788=ORIENTED_EDGE('',*,*,#48756,.F.);
#67789=ORIENTED_EDGE('',*,*,#50655,.F.);
#67790=ORIENTED_EDGE('',*,*,#46395,.F.);
#67791=ORIENTED_EDGE('',*,*,#48160,.F.);
#67792=ORIENTED_EDGE('',*,*,#48156,.T.);
#67793=ORIENTED_EDGE('',*,*,#50656,.F.);
#67794=ORIENTED_EDGE('',*,*,#48762,.F.);
#67795=ORIENTED_EDGE('',*,*,#50654,.T.);
#67796=ORIENTED_EDGE('',*,*,#50655,.T.);
#67797=ORIENTED_EDGE('',*,*,#50188,.F.);
#67798=ORIENTED_EDGE('',*,*,#50657,.F.);
#67799=ORIENTED_EDGE('',*,*,#46396,.F.);
#67800=ORIENTED_EDGE('',*,*,#50656,.T.);
#67801=ORIENTED_EDGE('',*,*,#48155,.F.);
#67802=ORIENTED_EDGE('',*,*,#50658,.F.);
#67803=ORIENTED_EDGE('',*,*,#48763,.F.);
#67804=ORIENTED_EDGE('',*,*,#50657,.T.);
#67805=ORIENTED_EDGE('',*,*,#48758,.F.);
#67806=ORIENTED_EDGE('',*,*,#50659,.F.);
#67807=ORIENTED_EDGE('',*,*,#46397,.F.);
#67808=ORIENTED_EDGE('',*,*,#50658,.T.);
#67809=ORIENTED_EDGE('',*,*,#48167,.F.);
#67810=ORIENTED_EDGE('',*,*,#50660,.F.);
#67811=ORIENTED_EDGE('',*,*,#48764,.F.);
#67812=ORIENTED_EDGE('',*,*,#50659,.T.);
#67813=ORIENTED_EDGE('',*,*,#48757,.F.);
#67814=ORIENTED_EDGE('',*,*,#50661,.F.);
#67815=ORIENTED_EDGE('',*,*,#48163,.F.);
#67816=ORIENTED_EDGE('',*,*,#50660,.T.);
#67817=ORIENTED_EDGE('',*,*,#48151,.F.);
#67818=ORIENTED_EDGE('',*,*,#50662,.F.);
#67819=ORIENTED_EDGE('',*,*,#48765,.F.);
#67820=ORIENTED_EDGE('',*,*,#50661,.T.);
#67821=ORIENTED_EDGE('',*,*,#48768,.F.);
#67822=ORIENTED_EDGE('',*,*,#50663,.F.);
#67823=ORIENTED_EDGE('',*,*,#48142,.F.);
#67824=ORIENTED_EDGE('',*,*,#50662,.T.);
#67825=ORIENTED_EDGE('',*,*,#48169,.F.);
#67826=ORIENTED_EDGE('',*,*,#50664,.F.);
#67827=ORIENTED_EDGE('',*,*,#48766,.F.);
#67828=ORIENTED_EDGE('',*,*,#50663,.T.);
#67829=ORIENTED_EDGE('',*,*,#48767,.F.);
#67830=ORIENTED_EDGE('',*,*,#50664,.T.);
#67831=ORIENTED_EDGE('',*,*,#48147,.F.);
#67832=ORIENTED_EDGE('',*,*,#48143,.T.);
#67833=ORIENTED_EDGE('',*,*,#50665,.F.);
#67834=ORIENTED_EDGE('',*,*,#48807,.F.);
#67835=ORIENTED_EDGE('',*,*,#50666,.F.);
#67836=ORIENTED_EDGE('',*,*,#48099,.F.);
#67837=ORIENTED_EDGE('',*,*,#50666,.T.);
#67838=ORIENTED_EDGE('',*,*,#48806,.F.);
#67839=ORIENTED_EDGE('',*,*,#50667,.F.);
#67840=ORIENTED_EDGE('',*,*,#48108,.F.);
#67841=ORIENTED_EDGE('',*,*,#48098,.T.);
#67842=ORIENTED_EDGE('',*,*,#48102,.F.);
#67843=ORIENTED_EDGE('',*,*,#50668,.F.);
#67844=ORIENTED_EDGE('',*,*,#48808,.F.);
#67845=ORIENTED_EDGE('',*,*,#50665,.T.);
#67846=ORIENTED_EDGE('',*,*,#50667,.T.);
#67847=ORIENTED_EDGE('',*,*,#48805,.F.);
#67848=ORIENTED_EDGE('',*,*,#50669,.F.);
#67849=ORIENTED_EDGE('',*,*,#48093,.F.);
#67850=ORIENTED_EDGE('',*,*,#50668,.T.);
#67851=ORIENTED_EDGE('',*,*,#48106,.F.);
#67852=ORIENTED_EDGE('',*,*,#50670,.F.);
#67853=ORIENTED_EDGE('',*,*,#48797,.F.);
#67854=ORIENTED_EDGE('',*,*,#50669,.T.);
#67855=ORIENTED_EDGE('',*,*,#48804,.F.);
#67856=ORIENTED_EDGE('',*,*,#50671,.F.);
#67857=ORIENTED_EDGE('',*,*,#48110,.F.);
#67858=ORIENTED_EDGE('',*,*,#50670,.T.);
#67859=ORIENTED_EDGE('',*,*,#45985,.F.);
#67860=ORIENTED_EDGE('',*,*,#50672,.F.);
#67861=ORIENTED_EDGE('',*,*,#48798,.F.);
#67862=ORIENTED_EDGE('',*,*,#50671,.T.);
#67863=ORIENTED_EDGE('',*,*,#48803,.F.);
#67864=ORIENTED_EDGE('',*,*,#50673,.F.);
#67865=ORIENTED_EDGE('',*,*,#48085,.T.);
#67866=ORIENTED_EDGE('',*,*,#48089,.F.);
#67867=ORIENTED_EDGE('',*,*,#50672,.T.);
#67868=ORIENTED_EDGE('',*,*,#45984,.F.);
#67869=ORIENTED_EDGE('',*,*,#50674,.F.);
#67870=ORIENTED_EDGE('',*,*,#50189,.F.);
#67871=ORIENTED_EDGE('',*,*,#50673,.T.);
#67872=ORIENTED_EDGE('',*,*,#48802,.F.);
#67873=ORIENTED_EDGE('',*,*,#50675,.F.);
#67874=ORIENTED_EDGE('',*,*,#48086,.F.);
#67875=ORIENTED_EDGE('',*,*,#50674,.T.);
#67876=ORIENTED_EDGE('',*,*,#45983,.F.);
#67877=ORIENTED_EDGE('',*,*,#50676,.F.);
#67878=ORIENTED_EDGE('',*,*,#48782,.F.);
#67879=ORIENTED_EDGE('',*,*,#50675,.T.);
#67880=ORIENTED_EDGE('',*,*,#48801,.F.);
#67881=ORIENTED_EDGE('',*,*,#50677,.F.);
#67882=ORIENTED_EDGE('',*,*,#48104,.F.);
#67883=ORIENTED_EDGE('',*,*,#50676,.T.);
#67884=ORIENTED_EDGE('',*,*,#45982,.F.);
#67885=ORIENTED_EDGE('',*,*,#50678,.F.);
#67886=ORIENTED_EDGE('',*,*,#50191,.F.);
#67887=ORIENTED_EDGE('',*,*,#50677,.T.);
#67888=ORIENTED_EDGE('',*,*,#48800,.F.);
#67889=ORIENTED_EDGE('',*,*,#50679,.F.);
#67890=ORIENTED_EDGE('',*,*,#46387,.F.);
#67891=ORIENTED_EDGE('',*,*,#50678,.T.);
#67892=ORIENTED_EDGE('',*,*,#45981,.F.);
#67893=ORIENTED_EDGE('',*,*,#50680,.F.);
#67894=ORIENTED_EDGE('',*,*,#48788,.F.);
#67895=ORIENTED_EDGE('',*,*,#50679,.T.);
#67896=ORIENTED_EDGE('',*,*,#50190,.F.);
#67897=ORIENTED_EDGE('',*,*,#50681,.F.);
#67898=ORIENTED_EDGE('',*,*,#46388,.F.);
#67899=ORIENTED_EDGE('',*,*,#50680,.T.);
#67900=ORIENTED_EDGE('',*,*,#48135,.F.);
#67901=ORIENTED_EDGE('',*,*,#50682,.F.);
#67902=ORIENTED_EDGE('',*,*,#48789,.F.);
#67903=ORIENTED_EDGE('',*,*,#50681,.T.);
#67904=ORIENTED_EDGE('',*,*,#48784,.F.);
#67905=ORIENTED_EDGE('',*,*,#50683,.F.);
#67906=ORIENTED_EDGE('',*,*,#46389,.F.);
#67907=ORIENTED_EDGE('',*,*,#48130,.F.);
#67908=ORIENTED_EDGE('',*,*,#48126,.T.);
#67909=ORIENTED_EDGE('',*,*,#50684,.F.);
#67910=ORIENTED_EDGE('',*,*,#48790,.F.);
#67911=ORIENTED_EDGE('',*,*,#50682,.T.);
#67912=ORIENTED_EDGE('',*,*,#50683,.T.);
#67913=ORIENTED_EDGE('',*,*,#50192,.F.);
#67914=ORIENTED_EDGE('',*,*,#50685,.F.);
#67915=ORIENTED_EDGE('',*,*,#46390,.F.);
#67916=ORIENTED_EDGE('',*,*,#50684,.T.);
#67917=ORIENTED_EDGE('',*,*,#48125,.F.);
#67918=ORIENTED_EDGE('',*,*,#50686,.F.);
#67919=ORIENTED_EDGE('',*,*,#48791,.F.);
#67920=ORIENTED_EDGE('',*,*,#50685,.T.);
#67921=ORIENTED_EDGE('',*,*,#48786,.F.);
#67922=ORIENTED_EDGE('',*,*,#50687,.F.);
#67923=ORIENTED_EDGE('',*,*,#46391,.F.);
#67924=ORIENTED_EDGE('',*,*,#50686,.T.);
#67925=ORIENTED_EDGE('',*,*,#48137,.F.);
#67926=ORIENTED_EDGE('',*,*,#50688,.F.);
#67927=ORIENTED_EDGE('',*,*,#48792,.F.);
#67928=ORIENTED_EDGE('',*,*,#50687,.T.);
#67929=ORIENTED_EDGE('',*,*,#48785,.F.);
#67930=ORIENTED_EDGE('',*,*,#50689,.F.);
#67931=ORIENTED_EDGE('',*,*,#48133,.F.);
#67932=ORIENTED_EDGE('',*,*,#50688,.T.);
#67933=ORIENTED_EDGE('',*,*,#48121,.F.);
#67934=ORIENTED_EDGE('',*,*,#50690,.F.);
#67935=ORIENTED_EDGE('',*,*,#48793,.F.);
#67936=ORIENTED_EDGE('',*,*,#50689,.T.);
#67937=ORIENTED_EDGE('',*,*,#48796,.F.);
#67938=ORIENTED_EDGE('',*,*,#50691,.F.);
#67939=ORIENTED_EDGE('',*,*,#48112,.F.);
#67940=ORIENTED_EDGE('',*,*,#50690,.T.);
#67941=ORIENTED_EDGE('',*,*,#48139,.F.);
#67942=ORIENTED_EDGE('',*,*,#50692,.F.);
#67943=ORIENTED_EDGE('',*,*,#48794,.F.);
#67944=ORIENTED_EDGE('',*,*,#50691,.T.);
#67945=ORIENTED_EDGE('',*,*,#48795,.F.);
#67946=ORIENTED_EDGE('',*,*,#50692,.T.);
#67947=ORIENTED_EDGE('',*,*,#48117,.F.);
#67948=ORIENTED_EDGE('',*,*,#48113,.T.);
#67949=ORIENTED_EDGE('',*,*,#50693,.F.);
#67950=ORIENTED_EDGE('',*,*,#48835,.F.);
#67951=ORIENTED_EDGE('',*,*,#50694,.F.);
#67952=ORIENTED_EDGE('',*,*,#48069,.F.);
#67953=ORIENTED_EDGE('',*,*,#50694,.T.);
#67954=ORIENTED_EDGE('',*,*,#48834,.F.);
#67955=ORIENTED_EDGE('',*,*,#50695,.F.);
#67956=ORIENTED_EDGE('',*,*,#48078,.F.);
#67957=ORIENTED_EDGE('',*,*,#48068,.T.);
#67958=ORIENTED_EDGE('',*,*,#48072,.F.);
#67959=ORIENTED_EDGE('',*,*,#50696,.F.);
#67960=ORIENTED_EDGE('',*,*,#48836,.F.);
#67961=ORIENTED_EDGE('',*,*,#50693,.T.);
#67962=ORIENTED_EDGE('',*,*,#50695,.T.);
#67963=ORIENTED_EDGE('',*,*,#48833,.F.);
#67964=ORIENTED_EDGE('',*,*,#50697,.F.);
#67965=ORIENTED_EDGE('',*,*,#48063,.F.);
#67966=ORIENTED_EDGE('',*,*,#50696,.T.);
#67967=ORIENTED_EDGE('',*,*,#48076,.F.);
#67968=ORIENTED_EDGE('',*,*,#50698,.F.);
#67969=ORIENTED_EDGE('',*,*,#48825,.F.);
#67970=ORIENTED_EDGE('',*,*,#50697,.T.);
#67971=ORIENTED_EDGE('',*,*,#48832,.F.);
#67972=ORIENTED_EDGE('',*,*,#50699,.F.);
#67973=ORIENTED_EDGE('',*,*,#48080,.F.);
#67974=ORIENTED_EDGE('',*,*,#50698,.T.);
#67975=ORIENTED_EDGE('',*,*,#45991,.F.);
#67976=ORIENTED_EDGE('',*,*,#50700,.F.);
#67977=ORIENTED_EDGE('',*,*,#48826,.F.);
#67978=ORIENTED_EDGE('',*,*,#50699,.T.);
#67979=ORIENTED_EDGE('',*,*,#48831,.F.);
#67980=ORIENTED_EDGE('',*,*,#50701,.F.);
#67981=ORIENTED_EDGE('',*,*,#48055,.T.);
#67982=ORIENTED_EDGE('',*,*,#48059,.F.);
#67983=ORIENTED_EDGE('',*,*,#50700,.T.);
#67984=ORIENTED_EDGE('',*,*,#45990,.F.);
#67985=ORIENTED_EDGE('',*,*,#50702,.F.);
#67986=ORIENTED_EDGE('',*,*,#50193,.F.);
#67987=ORIENTED_EDGE('',*,*,#50701,.T.);
#67988=ORIENTED_EDGE('',*,*,#48830,.F.);
#67989=ORIENTED_EDGE('',*,*,#50703,.F.);
#67990=ORIENTED_EDGE('',*,*,#48056,.F.);
#67991=ORIENTED_EDGE('',*,*,#50702,.T.);
#67992=ORIENTED_EDGE('',*,*,#45989,.F.);
#67993=ORIENTED_EDGE('',*,*,#50704,.F.);
#67994=ORIENTED_EDGE('',*,*,#48810,.F.);
#67995=ORIENTED_EDGE('',*,*,#50703,.T.);
#67996=ORIENTED_EDGE('',*,*,#48829,.F.);
#67997=ORIENTED_EDGE('',*,*,#50705,.F.);
#67998=ORIENTED_EDGE('',*,*,#48074,.F.);
#67999=ORIENTED_EDGE('',*,*,#50704,.T.);
#68000=ORIENTED_EDGE('',*,*,#45988,.F.);
#68001=ORIENTED_EDGE('',*,*,#50706,.F.);
#68002=ORIENTED_EDGE('',*,*,#50195,.F.);
#68003=ORIENTED_EDGE('',*,*,#50705,.T.);
#68004=ORIENTED_EDGE('',*,*,#48828,.F.);
#68005=ORIENTED_EDGE('',*,*,#50707,.F.);
#68006=ORIENTED_EDGE('',*,*,#46381,.F.);
#68007=ORIENTED_EDGE('',*,*,#50706,.T.);
#68008=ORIENTED_EDGE('',*,*,#45987,.F.);
#68009=ORIENTED_EDGE('',*,*,#50708,.F.);
#68010=ORIENTED_EDGE('',*,*,#48816,.F.);
#68011=ORIENTED_EDGE('',*,*,#50707,.T.);
#68012=ORIENTED_EDGE('',*,*,#50194,.F.);
#68013=ORIENTED_EDGE('',*,*,#50709,.F.);
#68014=ORIENTED_EDGE('',*,*,#46382,.F.);
#68015=ORIENTED_EDGE('',*,*,#50708,.T.);
#68016=ORIENTED_EDGE('',*,*,#48105,.F.);
#68017=ORIENTED_EDGE('',*,*,#50710,.F.);
#68018=ORIENTED_EDGE('',*,*,#48817,.F.);
#68019=ORIENTED_EDGE('',*,*,#50709,.T.);
#68020=ORIENTED_EDGE('',*,*,#48812,.F.);
#68021=ORIENTED_EDGE('',*,*,#50711,.F.);
#68022=ORIENTED_EDGE('',*,*,#46383,.F.);
#68023=ORIENTED_EDGE('',*,*,#48100,.F.);
#68024=ORIENTED_EDGE('',*,*,#48096,.T.);
#68025=ORIENTED_EDGE('',*,*,#50712,.F.);
#68026=ORIENTED_EDGE('',*,*,#48818,.F.);
#68027=ORIENTED_EDGE('',*,*,#50710,.T.);
#68028=ORIENTED_EDGE('',*,*,#50711,.T.);
#68029=ORIENTED_EDGE('',*,*,#50196,.F.);
#68030=ORIENTED_EDGE('',*,*,#50713,.F.);
#68031=ORIENTED_EDGE('',*,*,#46384,.F.);
#68032=ORIENTED_EDGE('',*,*,#50712,.T.);
#68033=ORIENTED_EDGE('',*,*,#48095,.F.);
#68034=ORIENTED_EDGE('',*,*,#50714,.F.);
#68035=ORIENTED_EDGE('',*,*,#48819,.F.);
#68036=ORIENTED_EDGE('',*,*,#50713,.T.);
#68037=ORIENTED_EDGE('',*,*,#48814,.F.);
#68038=ORIENTED_EDGE('',*,*,#50715,.F.);
#68039=ORIENTED_EDGE('',*,*,#46385,.F.);
#68040=ORIENTED_EDGE('',*,*,#50714,.T.);
#68041=ORIENTED_EDGE('',*,*,#48107,.F.);
#68042=ORIENTED_EDGE('',*,*,#50716,.F.);
#68043=ORIENTED_EDGE('',*,*,#48820,.F.);
#68044=ORIENTED_EDGE('',*,*,#50715,.T.);
#68045=ORIENTED_EDGE('',*,*,#48813,.F.);
#68046=ORIENTED_EDGE('',*,*,#50717,.F.);
#68047=ORIENTED_EDGE('',*,*,#48103,.F.);
#68048=ORIENTED_EDGE('',*,*,#50716,.T.);
#68049=ORIENTED_EDGE('',*,*,#48091,.F.);
#68050=ORIENTED_EDGE('',*,*,#50718,.F.);
#68051=ORIENTED_EDGE('',*,*,#48821,.F.);
#68052=ORIENTED_EDGE('',*,*,#50717,.T.);
#68053=ORIENTED_EDGE('',*,*,#48824,.F.);
#68054=ORIENTED_EDGE('',*,*,#50719,.F.);
#68055=ORIENTED_EDGE('',*,*,#48082,.F.);
#68056=ORIENTED_EDGE('',*,*,#50718,.T.);
#68057=ORIENTED_EDGE('',*,*,#48109,.F.);
#68058=ORIENTED_EDGE('',*,*,#50720,.F.);
#68059=ORIENTED_EDGE('',*,*,#48822,.F.);
#68060=ORIENTED_EDGE('',*,*,#50719,.T.);
#68061=ORIENTED_EDGE('',*,*,#48823,.F.);
#68062=ORIENTED_EDGE('',*,*,#50720,.T.);
#68063=ORIENTED_EDGE('',*,*,#48087,.F.);
#68064=ORIENTED_EDGE('',*,*,#48083,.T.);
#68065=ORIENTED_EDGE('',*,*,#50721,.F.);
#68066=ORIENTED_EDGE('',*,*,#48863,.F.);
#68067=ORIENTED_EDGE('',*,*,#50722,.F.);
#68068=ORIENTED_EDGE('',*,*,#48039,.F.);
#68069=ORIENTED_EDGE('',*,*,#50722,.T.);
#68070=ORIENTED_EDGE('',*,*,#48862,.F.);
#68071=ORIENTED_EDGE('',*,*,#50723,.F.);
#68072=ORIENTED_EDGE('',*,*,#48048,.F.);
#68073=ORIENTED_EDGE('',*,*,#48038,.T.);
#68074=ORIENTED_EDGE('',*,*,#48042,.F.);
#68075=ORIENTED_EDGE('',*,*,#50724,.F.);
#68076=ORIENTED_EDGE('',*,*,#48864,.F.);
#68077=ORIENTED_EDGE('',*,*,#50721,.T.);
#68078=ORIENTED_EDGE('',*,*,#50723,.T.);
#68079=ORIENTED_EDGE('',*,*,#48861,.F.);
#68080=ORIENTED_EDGE('',*,*,#50725,.F.);
#68081=ORIENTED_EDGE('',*,*,#48033,.F.);
#68082=ORIENTED_EDGE('',*,*,#50724,.T.);
#68083=ORIENTED_EDGE('',*,*,#48046,.F.);
#68084=ORIENTED_EDGE('',*,*,#50726,.F.);
#68085=ORIENTED_EDGE('',*,*,#48853,.F.);
#68086=ORIENTED_EDGE('',*,*,#50725,.T.);
#68087=ORIENTED_EDGE('',*,*,#48860,.F.);
#68088=ORIENTED_EDGE('',*,*,#50727,.F.);
#68089=ORIENTED_EDGE('',*,*,#48050,.F.);
#68090=ORIENTED_EDGE('',*,*,#50726,.T.);
#68091=ORIENTED_EDGE('',*,*,#45997,.F.);
#68092=ORIENTED_EDGE('',*,*,#50728,.F.);
#68093=ORIENTED_EDGE('',*,*,#48854,.F.);
#68094=ORIENTED_EDGE('',*,*,#50727,.T.);
#68095=ORIENTED_EDGE('',*,*,#48859,.F.);
#68096=ORIENTED_EDGE('',*,*,#50729,.F.);
#68097=ORIENTED_EDGE('',*,*,#48025,.T.);
#68098=ORIENTED_EDGE('',*,*,#48029,.F.);
#68099=ORIENTED_EDGE('',*,*,#50728,.T.);
#68100=ORIENTED_EDGE('',*,*,#45996,.F.);
#68101=ORIENTED_EDGE('',*,*,#50730,.F.);
#68102=ORIENTED_EDGE('',*,*,#50197,.F.);
#68103=ORIENTED_EDGE('',*,*,#50729,.T.);
#68104=ORIENTED_EDGE('',*,*,#48858,.F.);
#68105=ORIENTED_EDGE('',*,*,#50731,.F.);
#68106=ORIENTED_EDGE('',*,*,#48026,.F.);
#68107=ORIENTED_EDGE('',*,*,#50730,.T.);
#68108=ORIENTED_EDGE('',*,*,#45995,.F.);
#68109=ORIENTED_EDGE('',*,*,#50732,.F.);
#68110=ORIENTED_EDGE('',*,*,#48838,.F.);
#68111=ORIENTED_EDGE('',*,*,#50731,.T.);
#68112=ORIENTED_EDGE('',*,*,#48857,.F.);
#68113=ORIENTED_EDGE('',*,*,#50733,.F.);
#68114=ORIENTED_EDGE('',*,*,#48044,.F.);
#68115=ORIENTED_EDGE('',*,*,#50732,.T.);
#68116=ORIENTED_EDGE('',*,*,#45994,.F.);
#68117=ORIENTED_EDGE('',*,*,#50734,.F.);
#68118=ORIENTED_EDGE('',*,*,#50199,.F.);
#68119=ORIENTED_EDGE('',*,*,#50733,.T.);
#68120=ORIENTED_EDGE('',*,*,#48856,.F.);
#68121=ORIENTED_EDGE('',*,*,#50735,.F.);
#68122=ORIENTED_EDGE('',*,*,#46375,.F.);
#68123=ORIENTED_EDGE('',*,*,#50734,.T.);
#68124=ORIENTED_EDGE('',*,*,#45993,.F.);
#68125=ORIENTED_EDGE('',*,*,#50736,.F.);
#68126=ORIENTED_EDGE('',*,*,#48844,.F.);
#68127=ORIENTED_EDGE('',*,*,#50735,.T.);
#68128=ORIENTED_EDGE('',*,*,#50198,.F.);
#68129=ORIENTED_EDGE('',*,*,#50737,.F.);
#68130=ORIENTED_EDGE('',*,*,#46376,.F.);
#68131=ORIENTED_EDGE('',*,*,#50736,.T.);
#68132=ORIENTED_EDGE('',*,*,#48075,.F.);
#68133=ORIENTED_EDGE('',*,*,#50738,.F.);
#68134=ORIENTED_EDGE('',*,*,#48845,.F.);
#68135=ORIENTED_EDGE('',*,*,#50737,.T.);
#68136=ORIENTED_EDGE('',*,*,#48840,.F.);
#68137=ORIENTED_EDGE('',*,*,#50739,.F.);
#68138=ORIENTED_EDGE('',*,*,#46377,.F.);
#68139=ORIENTED_EDGE('',*,*,#48070,.F.);
#68140=ORIENTED_EDGE('',*,*,#48066,.T.);
#68141=ORIENTED_EDGE('',*,*,#50740,.F.);
#68142=ORIENTED_EDGE('',*,*,#48846,.F.);
#68143=ORIENTED_EDGE('',*,*,#50738,.T.);
#68144=ORIENTED_EDGE('',*,*,#50739,.T.);
#68145=ORIENTED_EDGE('',*,*,#50200,.F.);
#68146=ORIENTED_EDGE('',*,*,#50741,.F.);
#68147=ORIENTED_EDGE('',*,*,#46378,.F.);
#68148=ORIENTED_EDGE('',*,*,#50740,.T.);
#68149=ORIENTED_EDGE('',*,*,#48065,.F.);
#68150=ORIENTED_EDGE('',*,*,#50742,.F.);
#68151=ORIENTED_EDGE('',*,*,#48847,.F.);
#68152=ORIENTED_EDGE('',*,*,#50741,.T.);
#68153=ORIENTED_EDGE('',*,*,#48842,.F.);
#68154=ORIENTED_EDGE('',*,*,#50743,.F.);
#68155=ORIENTED_EDGE('',*,*,#46379,.F.);
#68156=ORIENTED_EDGE('',*,*,#50742,.T.);
#68157=ORIENTED_EDGE('',*,*,#48077,.F.);
#68158=ORIENTED_EDGE('',*,*,#50744,.F.);
#68159=ORIENTED_EDGE('',*,*,#48848,.F.);
#68160=ORIENTED_EDGE('',*,*,#50743,.T.);
#68161=ORIENTED_EDGE('',*,*,#48841,.F.);
#68162=ORIENTED_EDGE('',*,*,#50745,.F.);
#68163=ORIENTED_EDGE('',*,*,#48073,.F.);
#68164=ORIENTED_EDGE('',*,*,#50744,.T.);
#68165=ORIENTED_EDGE('',*,*,#48061,.F.);
#68166=ORIENTED_EDGE('',*,*,#50746,.F.);
#68167=ORIENTED_EDGE('',*,*,#48849,.F.);
#68168=ORIENTED_EDGE('',*,*,#50745,.T.);
#68169=ORIENTED_EDGE('',*,*,#48852,.F.);
#68170=ORIENTED_EDGE('',*,*,#50747,.F.);
#68171=ORIENTED_EDGE('',*,*,#48052,.F.);
#68172=ORIENTED_EDGE('',*,*,#50746,.T.);
#68173=ORIENTED_EDGE('',*,*,#48079,.F.);
#68174=ORIENTED_EDGE('',*,*,#50748,.F.);
#68175=ORIENTED_EDGE('',*,*,#48850,.F.);
#68176=ORIENTED_EDGE('',*,*,#50747,.T.);
#68177=ORIENTED_EDGE('',*,*,#48851,.F.);
#68178=ORIENTED_EDGE('',*,*,#50748,.T.);
#68179=ORIENTED_EDGE('',*,*,#48057,.F.);
#68180=ORIENTED_EDGE('',*,*,#48053,.T.);
#68181=ORIENTED_EDGE('',*,*,#50749,.F.);
#68182=ORIENTED_EDGE('',*,*,#48891,.F.);
#68183=ORIENTED_EDGE('',*,*,#50750,.F.);
#68184=ORIENTED_EDGE('',*,*,#48009,.F.);
#68185=ORIENTED_EDGE('',*,*,#50750,.T.);
#68186=ORIENTED_EDGE('',*,*,#48890,.F.);
#68187=ORIENTED_EDGE('',*,*,#50751,.F.);
#68188=ORIENTED_EDGE('',*,*,#48018,.F.);
#68189=ORIENTED_EDGE('',*,*,#48008,.T.);
#68190=ORIENTED_EDGE('',*,*,#48012,.F.);
#68191=ORIENTED_EDGE('',*,*,#50752,.F.);
#68192=ORIENTED_EDGE('',*,*,#48892,.F.);
#68193=ORIENTED_EDGE('',*,*,#50749,.T.);
#68194=ORIENTED_EDGE('',*,*,#50751,.T.);
#68195=ORIENTED_EDGE('',*,*,#48889,.F.);
#68196=ORIENTED_EDGE('',*,*,#50753,.F.);
#68197=ORIENTED_EDGE('',*,*,#48003,.F.);
#68198=ORIENTED_EDGE('',*,*,#50752,.T.);
#68199=ORIENTED_EDGE('',*,*,#48016,.F.);
#68200=ORIENTED_EDGE('',*,*,#50754,.F.);
#68201=ORIENTED_EDGE('',*,*,#48881,.F.);
#68202=ORIENTED_EDGE('',*,*,#50753,.T.);
#68203=ORIENTED_EDGE('',*,*,#48888,.F.);
#68204=ORIENTED_EDGE('',*,*,#50755,.F.);
#68205=ORIENTED_EDGE('',*,*,#48020,.F.);
#68206=ORIENTED_EDGE('',*,*,#50754,.T.);
#68207=ORIENTED_EDGE('',*,*,#46003,.F.);
#68208=ORIENTED_EDGE('',*,*,#50756,.F.);
#68209=ORIENTED_EDGE('',*,*,#48882,.F.);
#68210=ORIENTED_EDGE('',*,*,#50755,.T.);
#68211=ORIENTED_EDGE('',*,*,#48887,.F.);
#68212=ORIENTED_EDGE('',*,*,#50757,.F.);
#68213=ORIENTED_EDGE('',*,*,#47995,.T.);
#68214=ORIENTED_EDGE('',*,*,#47999,.F.);
#68215=ORIENTED_EDGE('',*,*,#50756,.T.);
#68216=ORIENTED_EDGE('',*,*,#46002,.F.);
#68217=ORIENTED_EDGE('',*,*,#50758,.F.);
#68218=ORIENTED_EDGE('',*,*,#50201,.F.);
#68219=ORIENTED_EDGE('',*,*,#50757,.T.);
#68220=ORIENTED_EDGE('',*,*,#48886,.F.);
#68221=ORIENTED_EDGE('',*,*,#50759,.F.);
#68222=ORIENTED_EDGE('',*,*,#47996,.F.);
#68223=ORIENTED_EDGE('',*,*,#50758,.T.);
#68224=ORIENTED_EDGE('',*,*,#46001,.F.);
#68225=ORIENTED_EDGE('',*,*,#50760,.F.);
#68226=ORIENTED_EDGE('',*,*,#48866,.F.);
#68227=ORIENTED_EDGE('',*,*,#50759,.T.);
#68228=ORIENTED_EDGE('',*,*,#48885,.F.);
#68229=ORIENTED_EDGE('',*,*,#50761,.F.);
#68230=ORIENTED_EDGE('',*,*,#48014,.F.);
#68231=ORIENTED_EDGE('',*,*,#50760,.T.);
#68232=ORIENTED_EDGE('',*,*,#46000,.F.);
#68233=ORIENTED_EDGE('',*,*,#50762,.F.);
#68234=ORIENTED_EDGE('',*,*,#50203,.F.);
#68235=ORIENTED_EDGE('',*,*,#50761,.T.);
#68236=ORIENTED_EDGE('',*,*,#48884,.F.);
#68237=ORIENTED_EDGE('',*,*,#50763,.F.);
#68238=ORIENTED_EDGE('',*,*,#46369,.F.);
#68239=ORIENTED_EDGE('',*,*,#50762,.T.);
#68240=ORIENTED_EDGE('',*,*,#45999,.F.);
#68241=ORIENTED_EDGE('',*,*,#50764,.F.);
#68242=ORIENTED_EDGE('',*,*,#48872,.F.);
#68243=ORIENTED_EDGE('',*,*,#50763,.T.);
#68244=ORIENTED_EDGE('',*,*,#50202,.F.);
#68245=ORIENTED_EDGE('',*,*,#50765,.F.);
#68246=ORIENTED_EDGE('',*,*,#46370,.F.);
#68247=ORIENTED_EDGE('',*,*,#50764,.T.);
#68248=ORIENTED_EDGE('',*,*,#48045,.F.);
#68249=ORIENTED_EDGE('',*,*,#50766,.F.);
#68250=ORIENTED_EDGE('',*,*,#48873,.F.);
#68251=ORIENTED_EDGE('',*,*,#50765,.T.);
#68252=ORIENTED_EDGE('',*,*,#48868,.F.);
#68253=ORIENTED_EDGE('',*,*,#50767,.F.);
#68254=ORIENTED_EDGE('',*,*,#46371,.F.);
#68255=ORIENTED_EDGE('',*,*,#48040,.F.);
#68256=ORIENTED_EDGE('',*,*,#48036,.T.);
#68257=ORIENTED_EDGE('',*,*,#50768,.F.);
#68258=ORIENTED_EDGE('',*,*,#48874,.F.);
#68259=ORIENTED_EDGE('',*,*,#50766,.T.);
#68260=ORIENTED_EDGE('',*,*,#50767,.T.);
#68261=ORIENTED_EDGE('',*,*,#50204,.F.);
#68262=ORIENTED_EDGE('',*,*,#50769,.F.);
#68263=ORIENTED_EDGE('',*,*,#46372,.F.);
#68264=ORIENTED_EDGE('',*,*,#50768,.T.);
#68265=ORIENTED_EDGE('',*,*,#48035,.F.);
#68266=ORIENTED_EDGE('',*,*,#50770,.F.);
#68267=ORIENTED_EDGE('',*,*,#48875,.F.);
#68268=ORIENTED_EDGE('',*,*,#50769,.T.);
#68269=ORIENTED_EDGE('',*,*,#48870,.F.);
#68270=ORIENTED_EDGE('',*,*,#50771,.F.);
#68271=ORIENTED_EDGE('',*,*,#46373,.F.);
#68272=ORIENTED_EDGE('',*,*,#50770,.T.);
#68273=ORIENTED_EDGE('',*,*,#48047,.F.);
#68274=ORIENTED_EDGE('',*,*,#50772,.F.);
#68275=ORIENTED_EDGE('',*,*,#48876,.F.);
#68276=ORIENTED_EDGE('',*,*,#50771,.T.);
#68277=ORIENTED_EDGE('',*,*,#48869,.F.);
#68278=ORIENTED_EDGE('',*,*,#50773,.F.);
#68279=ORIENTED_EDGE('',*,*,#48043,.F.);
#68280=ORIENTED_EDGE('',*,*,#50772,.T.);
#68281=ORIENTED_EDGE('',*,*,#48031,.F.);
#68282=ORIENTED_EDGE('',*,*,#50774,.F.);
#68283=ORIENTED_EDGE('',*,*,#48877,.F.);
#68284=ORIENTED_EDGE('',*,*,#50773,.T.);
#68285=ORIENTED_EDGE('',*,*,#48880,.F.);
#68286=ORIENTED_EDGE('',*,*,#50775,.F.);
#68287=ORIENTED_EDGE('',*,*,#48022,.F.);
#68288=ORIENTED_EDGE('',*,*,#50774,.T.);
#68289=ORIENTED_EDGE('',*,*,#48049,.F.);
#68290=ORIENTED_EDGE('',*,*,#50776,.F.);
#68291=ORIENTED_EDGE('',*,*,#48878,.F.);
#68292=ORIENTED_EDGE('',*,*,#50775,.T.);
#68293=ORIENTED_EDGE('',*,*,#48879,.F.);
#68294=ORIENTED_EDGE('',*,*,#50776,.T.);
#68295=ORIENTED_EDGE('',*,*,#48027,.F.);
#68296=ORIENTED_EDGE('',*,*,#48023,.T.);
#68297=ORIENTED_EDGE('',*,*,#50777,.F.);
#68298=ORIENTED_EDGE('',*,*,#48919,.F.);
#68299=ORIENTED_EDGE('',*,*,#50778,.F.);
#68300=ORIENTED_EDGE('',*,*,#47979,.F.);
#68301=ORIENTED_EDGE('',*,*,#50778,.T.);
#68302=ORIENTED_EDGE('',*,*,#48918,.F.);
#68303=ORIENTED_EDGE('',*,*,#50779,.F.);
#68304=ORIENTED_EDGE('',*,*,#47988,.F.);
#68305=ORIENTED_EDGE('',*,*,#47978,.T.);
#68306=ORIENTED_EDGE('',*,*,#47982,.F.);
#68307=ORIENTED_EDGE('',*,*,#50780,.F.);
#68308=ORIENTED_EDGE('',*,*,#48920,.F.);
#68309=ORIENTED_EDGE('',*,*,#50777,.T.);
#68310=ORIENTED_EDGE('',*,*,#50779,.T.);
#68311=ORIENTED_EDGE('',*,*,#48917,.F.);
#68312=ORIENTED_EDGE('',*,*,#50781,.F.);
#68313=ORIENTED_EDGE('',*,*,#47973,.F.);
#68314=ORIENTED_EDGE('',*,*,#50780,.T.);
#68315=ORIENTED_EDGE('',*,*,#47986,.F.);
#68316=ORIENTED_EDGE('',*,*,#50782,.F.);
#68317=ORIENTED_EDGE('',*,*,#48909,.F.);
#68318=ORIENTED_EDGE('',*,*,#50781,.T.);
#68319=ORIENTED_EDGE('',*,*,#48916,.F.);
#68320=ORIENTED_EDGE('',*,*,#50783,.F.);
#68321=ORIENTED_EDGE('',*,*,#47990,.F.);
#68322=ORIENTED_EDGE('',*,*,#50782,.T.);
#68323=ORIENTED_EDGE('',*,*,#46009,.F.);
#68324=ORIENTED_EDGE('',*,*,#50784,.F.);
#68325=ORIENTED_EDGE('',*,*,#48910,.F.);
#68326=ORIENTED_EDGE('',*,*,#50783,.T.);
#68327=ORIENTED_EDGE('',*,*,#48915,.F.);
#68328=ORIENTED_EDGE('',*,*,#50785,.F.);
#68329=ORIENTED_EDGE('',*,*,#47965,.T.);
#68330=ORIENTED_EDGE('',*,*,#47969,.F.);
#68331=ORIENTED_EDGE('',*,*,#50784,.T.);
#68332=ORIENTED_EDGE('',*,*,#46008,.F.);
#68333=ORIENTED_EDGE('',*,*,#50786,.F.);
#68334=ORIENTED_EDGE('',*,*,#50205,.F.);
#68335=ORIENTED_EDGE('',*,*,#50785,.T.);
#68336=ORIENTED_EDGE('',*,*,#48914,.F.);
#68337=ORIENTED_EDGE('',*,*,#50787,.F.);
#68338=ORIENTED_EDGE('',*,*,#47966,.F.);
#68339=ORIENTED_EDGE('',*,*,#50786,.T.);
#68340=ORIENTED_EDGE('',*,*,#46007,.F.);
#68341=ORIENTED_EDGE('',*,*,#50788,.F.);
#68342=ORIENTED_EDGE('',*,*,#48894,.F.);
#68343=ORIENTED_EDGE('',*,*,#50787,.T.);
#68344=ORIENTED_EDGE('',*,*,#48913,.F.);
#68345=ORIENTED_EDGE('',*,*,#50789,.F.);
#68346=ORIENTED_EDGE('',*,*,#47984,.F.);
#68347=ORIENTED_EDGE('',*,*,#50788,.T.);
#68348=ORIENTED_EDGE('',*,*,#46006,.F.);
#68349=ORIENTED_EDGE('',*,*,#50790,.F.);
#68350=ORIENTED_EDGE('',*,*,#50207,.F.);
#68351=ORIENTED_EDGE('',*,*,#50789,.T.);
#68352=ORIENTED_EDGE('',*,*,#48912,.F.);
#68353=ORIENTED_EDGE('',*,*,#50791,.F.);
#68354=ORIENTED_EDGE('',*,*,#46363,.F.);
#68355=ORIENTED_EDGE('',*,*,#50790,.T.);
#68356=ORIENTED_EDGE('',*,*,#46005,.F.);
#68357=ORIENTED_EDGE('',*,*,#50792,.F.);
#68358=ORIENTED_EDGE('',*,*,#48900,.F.);
#68359=ORIENTED_EDGE('',*,*,#50791,.T.);
#68360=ORIENTED_EDGE('',*,*,#50206,.F.);
#68361=ORIENTED_EDGE('',*,*,#50793,.F.);
#68362=ORIENTED_EDGE('',*,*,#46364,.F.);
#68363=ORIENTED_EDGE('',*,*,#50792,.T.);
#68364=ORIENTED_EDGE('',*,*,#48015,.F.);
#68365=ORIENTED_EDGE('',*,*,#50794,.F.);
#68366=ORIENTED_EDGE('',*,*,#48901,.F.);
#68367=ORIENTED_EDGE('',*,*,#50793,.T.);
#68368=ORIENTED_EDGE('',*,*,#48896,.F.);
#68369=ORIENTED_EDGE('',*,*,#50795,.F.);
#68370=ORIENTED_EDGE('',*,*,#46365,.F.);
#68371=ORIENTED_EDGE('',*,*,#48010,.F.);
#68372=ORIENTED_EDGE('',*,*,#48006,.T.);
#68373=ORIENTED_EDGE('',*,*,#50796,.F.);
#68374=ORIENTED_EDGE('',*,*,#48902,.F.);
#68375=ORIENTED_EDGE('',*,*,#50794,.T.);
#68376=ORIENTED_EDGE('',*,*,#50795,.T.);
#68377=ORIENTED_EDGE('',*,*,#50208,.F.);
#68378=ORIENTED_EDGE('',*,*,#50797,.F.);
#68379=ORIENTED_EDGE('',*,*,#46366,.F.);
#68380=ORIENTED_EDGE('',*,*,#50796,.T.);
#68381=ORIENTED_EDGE('',*,*,#48005,.F.);
#68382=ORIENTED_EDGE('',*,*,#50798,.F.);
#68383=ORIENTED_EDGE('',*,*,#48903,.F.);
#68384=ORIENTED_EDGE('',*,*,#50797,.T.);
#68385=ORIENTED_EDGE('',*,*,#48898,.F.);
#68386=ORIENTED_EDGE('',*,*,#50799,.F.);
#68387=ORIENTED_EDGE('',*,*,#46367,.F.);
#68388=ORIENTED_EDGE('',*,*,#50798,.T.);
#68389=ORIENTED_EDGE('',*,*,#48017,.F.);
#68390=ORIENTED_EDGE('',*,*,#50800,.F.);
#68391=ORIENTED_EDGE('',*,*,#48904,.F.);
#68392=ORIENTED_EDGE('',*,*,#50799,.T.);
#68393=ORIENTED_EDGE('',*,*,#48897,.F.);
#68394=ORIENTED_EDGE('',*,*,#50801,.F.);
#68395=ORIENTED_EDGE('',*,*,#48013,.F.);
#68396=ORIENTED_EDGE('',*,*,#50800,.T.);
#68397=ORIENTED_EDGE('',*,*,#48001,.F.);
#68398=ORIENTED_EDGE('',*,*,#50802,.F.);
#68399=ORIENTED_EDGE('',*,*,#48905,.F.);
#68400=ORIENTED_EDGE('',*,*,#50801,.T.);
#68401=ORIENTED_EDGE('',*,*,#48908,.F.);
#68402=ORIENTED_EDGE('',*,*,#50803,.F.);
#68403=ORIENTED_EDGE('',*,*,#47992,.F.);
#68404=ORIENTED_EDGE('',*,*,#50802,.T.);
#68405=ORIENTED_EDGE('',*,*,#48019,.F.);
#68406=ORIENTED_EDGE('',*,*,#50804,.F.);
#68407=ORIENTED_EDGE('',*,*,#48906,.F.);
#68408=ORIENTED_EDGE('',*,*,#50803,.T.);
#68409=ORIENTED_EDGE('',*,*,#48907,.F.);
#68410=ORIENTED_EDGE('',*,*,#50804,.T.);
#68411=ORIENTED_EDGE('',*,*,#47997,.F.);
#68412=ORIENTED_EDGE('',*,*,#47993,.T.);
#68413=ORIENTED_EDGE('',*,*,#50805,.F.);
#68414=ORIENTED_EDGE('',*,*,#48947,.F.);
#68415=ORIENTED_EDGE('',*,*,#50806,.F.);
#68416=ORIENTED_EDGE('',*,*,#47949,.F.);
#68417=ORIENTED_EDGE('',*,*,#50806,.T.);
#68418=ORIENTED_EDGE('',*,*,#48946,.F.);
#68419=ORIENTED_EDGE('',*,*,#50807,.F.);
#68420=ORIENTED_EDGE('',*,*,#47958,.F.);
#68421=ORIENTED_EDGE('',*,*,#47948,.T.);
#68422=ORIENTED_EDGE('',*,*,#47952,.F.);
#68423=ORIENTED_EDGE('',*,*,#50808,.F.);
#68424=ORIENTED_EDGE('',*,*,#48948,.F.);
#68425=ORIENTED_EDGE('',*,*,#50805,.T.);
#68426=ORIENTED_EDGE('',*,*,#50807,.T.);
#68427=ORIENTED_EDGE('',*,*,#48945,.F.);
#68428=ORIENTED_EDGE('',*,*,#50809,.F.);
#68429=ORIENTED_EDGE('',*,*,#47943,.F.);
#68430=ORIENTED_EDGE('',*,*,#50808,.T.);
#68431=ORIENTED_EDGE('',*,*,#47956,.F.);
#68432=ORIENTED_EDGE('',*,*,#50810,.F.);
#68433=ORIENTED_EDGE('',*,*,#48937,.F.);
#68434=ORIENTED_EDGE('',*,*,#50809,.T.);
#68435=ORIENTED_EDGE('',*,*,#48944,.F.);
#68436=ORIENTED_EDGE('',*,*,#50811,.F.);
#68437=ORIENTED_EDGE('',*,*,#47960,.F.);
#68438=ORIENTED_EDGE('',*,*,#50810,.T.);
#68439=ORIENTED_EDGE('',*,*,#46015,.F.);
#68440=ORIENTED_EDGE('',*,*,#50812,.F.);
#68441=ORIENTED_EDGE('',*,*,#48938,.F.);
#68442=ORIENTED_EDGE('',*,*,#50811,.T.);
#68443=ORIENTED_EDGE('',*,*,#48943,.F.);
#68444=ORIENTED_EDGE('',*,*,#50813,.F.);
#68445=ORIENTED_EDGE('',*,*,#47935,.T.);
#68446=ORIENTED_EDGE('',*,*,#47939,.F.);
#68447=ORIENTED_EDGE('',*,*,#50812,.T.);
#68448=ORIENTED_EDGE('',*,*,#46014,.F.);
#68449=ORIENTED_EDGE('',*,*,#50814,.F.);
#68450=ORIENTED_EDGE('',*,*,#50209,.F.);
#68451=ORIENTED_EDGE('',*,*,#50813,.T.);
#68452=ORIENTED_EDGE('',*,*,#48942,.F.);
#68453=ORIENTED_EDGE('',*,*,#50815,.F.);
#68454=ORIENTED_EDGE('',*,*,#47936,.F.);
#68455=ORIENTED_EDGE('',*,*,#50814,.T.);
#68456=ORIENTED_EDGE('',*,*,#46013,.F.);
#68457=ORIENTED_EDGE('',*,*,#50816,.F.);
#68458=ORIENTED_EDGE('',*,*,#48922,.F.);
#68459=ORIENTED_EDGE('',*,*,#50815,.T.);
#68460=ORIENTED_EDGE('',*,*,#48941,.F.);
#68461=ORIENTED_EDGE('',*,*,#50817,.F.);
#68462=ORIENTED_EDGE('',*,*,#47954,.F.);
#68463=ORIENTED_EDGE('',*,*,#50816,.T.);
#68464=ORIENTED_EDGE('',*,*,#46012,.F.);
#68465=ORIENTED_EDGE('',*,*,#50818,.F.);
#68466=ORIENTED_EDGE('',*,*,#50211,.F.);
#68467=ORIENTED_EDGE('',*,*,#50817,.T.);
#68468=ORIENTED_EDGE('',*,*,#48940,.F.);
#68469=ORIENTED_EDGE('',*,*,#50819,.F.);
#68470=ORIENTED_EDGE('',*,*,#46357,.F.);
#68471=ORIENTED_EDGE('',*,*,#50818,.T.);
#68472=ORIENTED_EDGE('',*,*,#46011,.F.);
#68473=ORIENTED_EDGE('',*,*,#50820,.F.);
#68474=ORIENTED_EDGE('',*,*,#48928,.F.);
#68475=ORIENTED_EDGE('',*,*,#50819,.T.);
#68476=ORIENTED_EDGE('',*,*,#50210,.F.);
#68477=ORIENTED_EDGE('',*,*,#50821,.F.);
#68478=ORIENTED_EDGE('',*,*,#46358,.F.);
#68479=ORIENTED_EDGE('',*,*,#50820,.T.);
#68480=ORIENTED_EDGE('',*,*,#47985,.F.);
#68481=ORIENTED_EDGE('',*,*,#50822,.F.);
#68482=ORIENTED_EDGE('',*,*,#48929,.F.);
#68483=ORIENTED_EDGE('',*,*,#50821,.T.);
#68484=ORIENTED_EDGE('',*,*,#48924,.F.);
#68485=ORIENTED_EDGE('',*,*,#50823,.F.);
#68486=ORIENTED_EDGE('',*,*,#46359,.F.);
#68487=ORIENTED_EDGE('',*,*,#47980,.F.);
#68488=ORIENTED_EDGE('',*,*,#47976,.T.);
#68489=ORIENTED_EDGE('',*,*,#50824,.F.);
#68490=ORIENTED_EDGE('',*,*,#48930,.F.);
#68491=ORIENTED_EDGE('',*,*,#50822,.T.);
#68492=ORIENTED_EDGE('',*,*,#50823,.T.);
#68493=ORIENTED_EDGE('',*,*,#50212,.F.);
#68494=ORIENTED_EDGE('',*,*,#50825,.F.);
#68495=ORIENTED_EDGE('',*,*,#46360,.F.);
#68496=ORIENTED_EDGE('',*,*,#50824,.T.);
#68497=ORIENTED_EDGE('',*,*,#47975,.F.);
#68498=ORIENTED_EDGE('',*,*,#50826,.F.);
#68499=ORIENTED_EDGE('',*,*,#48931,.F.);
#68500=ORIENTED_EDGE('',*,*,#50825,.T.);
#68501=ORIENTED_EDGE('',*,*,#48926,.F.);
#68502=ORIENTED_EDGE('',*,*,#50827,.F.);
#68503=ORIENTED_EDGE('',*,*,#46361,.F.);
#68504=ORIENTED_EDGE('',*,*,#50826,.T.);
#68505=ORIENTED_EDGE('',*,*,#47987,.F.);
#68506=ORIENTED_EDGE('',*,*,#50828,.F.);
#68507=ORIENTED_EDGE('',*,*,#48932,.F.);
#68508=ORIENTED_EDGE('',*,*,#50827,.T.);
#68509=ORIENTED_EDGE('',*,*,#48925,.F.);
#68510=ORIENTED_EDGE('',*,*,#50829,.F.);
#68511=ORIENTED_EDGE('',*,*,#47983,.F.);
#68512=ORIENTED_EDGE('',*,*,#50828,.T.);
#68513=ORIENTED_EDGE('',*,*,#47971,.F.);
#68514=ORIENTED_EDGE('',*,*,#50830,.F.);
#68515=ORIENTED_EDGE('',*,*,#48933,.F.);
#68516=ORIENTED_EDGE('',*,*,#50829,.T.);
#68517=ORIENTED_EDGE('',*,*,#48936,.F.);
#68518=ORIENTED_EDGE('',*,*,#50831,.F.);
#68519=ORIENTED_EDGE('',*,*,#47962,.F.);
#68520=ORIENTED_EDGE('',*,*,#50830,.T.);
#68521=ORIENTED_EDGE('',*,*,#47989,.F.);
#68522=ORIENTED_EDGE('',*,*,#50832,.F.);
#68523=ORIENTED_EDGE('',*,*,#48934,.F.);
#68524=ORIENTED_EDGE('',*,*,#50831,.T.);
#68525=ORIENTED_EDGE('',*,*,#48935,.F.);
#68526=ORIENTED_EDGE('',*,*,#50832,.T.);
#68527=ORIENTED_EDGE('',*,*,#47967,.F.);
#68528=ORIENTED_EDGE('',*,*,#47963,.T.);
#68529=ORIENTED_EDGE('',*,*,#50833,.F.);
#68530=ORIENTED_EDGE('',*,*,#48975,.F.);
#68531=ORIENTED_EDGE('',*,*,#50834,.F.);
#68532=ORIENTED_EDGE('',*,*,#47919,.F.);
#68533=ORIENTED_EDGE('',*,*,#50834,.T.);
#68534=ORIENTED_EDGE('',*,*,#48974,.F.);
#68535=ORIENTED_EDGE('',*,*,#50835,.F.);
#68536=ORIENTED_EDGE('',*,*,#47928,.F.);
#68537=ORIENTED_EDGE('',*,*,#47918,.T.);
#68538=ORIENTED_EDGE('',*,*,#47922,.F.);
#68539=ORIENTED_EDGE('',*,*,#50836,.F.);
#68540=ORIENTED_EDGE('',*,*,#48976,.F.);
#68541=ORIENTED_EDGE('',*,*,#50833,.T.);
#68542=ORIENTED_EDGE('',*,*,#50835,.T.);
#68543=ORIENTED_EDGE('',*,*,#48973,.F.);
#68544=ORIENTED_EDGE('',*,*,#50837,.F.);
#68545=ORIENTED_EDGE('',*,*,#47913,.F.);
#68546=ORIENTED_EDGE('',*,*,#50836,.T.);
#68547=ORIENTED_EDGE('',*,*,#47926,.F.);
#68548=ORIENTED_EDGE('',*,*,#50838,.F.);
#68549=ORIENTED_EDGE('',*,*,#48965,.F.);
#68550=ORIENTED_EDGE('',*,*,#50837,.T.);
#68551=ORIENTED_EDGE('',*,*,#48972,.F.);
#68552=ORIENTED_EDGE('',*,*,#50839,.F.);
#68553=ORIENTED_EDGE('',*,*,#47930,.F.);
#68554=ORIENTED_EDGE('',*,*,#50838,.T.);
#68555=ORIENTED_EDGE('',*,*,#46021,.F.);
#68556=ORIENTED_EDGE('',*,*,#50840,.F.);
#68557=ORIENTED_EDGE('',*,*,#48966,.F.);
#68558=ORIENTED_EDGE('',*,*,#50839,.T.);
#68559=ORIENTED_EDGE('',*,*,#48971,.F.);
#68560=ORIENTED_EDGE('',*,*,#50841,.F.);
#68561=ORIENTED_EDGE('',*,*,#47905,.T.);
#68562=ORIENTED_EDGE('',*,*,#47909,.F.);
#68563=ORIENTED_EDGE('',*,*,#50840,.T.);
#68564=ORIENTED_EDGE('',*,*,#46020,.F.);
#68565=ORIENTED_EDGE('',*,*,#50842,.F.);
#68566=ORIENTED_EDGE('',*,*,#50213,.F.);
#68567=ORIENTED_EDGE('',*,*,#50841,.T.);
#68568=ORIENTED_EDGE('',*,*,#48970,.F.);
#68569=ORIENTED_EDGE('',*,*,#50843,.F.);
#68570=ORIENTED_EDGE('',*,*,#47906,.F.);
#68571=ORIENTED_EDGE('',*,*,#50842,.T.);
#68572=ORIENTED_EDGE('',*,*,#46019,.F.);
#68573=ORIENTED_EDGE('',*,*,#50844,.F.);
#68574=ORIENTED_EDGE('',*,*,#48950,.F.);
#68575=ORIENTED_EDGE('',*,*,#50843,.T.);
#68576=ORIENTED_EDGE('',*,*,#48969,.F.);
#68577=ORIENTED_EDGE('',*,*,#50845,.F.);
#68578=ORIENTED_EDGE('',*,*,#47924,.F.);
#68579=ORIENTED_EDGE('',*,*,#50844,.T.);
#68580=ORIENTED_EDGE('',*,*,#46018,.F.);
#68581=ORIENTED_EDGE('',*,*,#50846,.F.);
#68582=ORIENTED_EDGE('',*,*,#50215,.F.);
#68583=ORIENTED_EDGE('',*,*,#50845,.T.);
#68584=ORIENTED_EDGE('',*,*,#48968,.F.);
#68585=ORIENTED_EDGE('',*,*,#50847,.F.);
#68586=ORIENTED_EDGE('',*,*,#46351,.F.);
#68587=ORIENTED_EDGE('',*,*,#50846,.T.);
#68588=ORIENTED_EDGE('',*,*,#46017,.F.);
#68589=ORIENTED_EDGE('',*,*,#50848,.F.);
#68590=ORIENTED_EDGE('',*,*,#48956,.F.);
#68591=ORIENTED_EDGE('',*,*,#50847,.T.);
#68592=ORIENTED_EDGE('',*,*,#50214,.F.);
#68593=ORIENTED_EDGE('',*,*,#50849,.F.);
#68594=ORIENTED_EDGE('',*,*,#46352,.F.);
#68595=ORIENTED_EDGE('',*,*,#50848,.T.);
#68596=ORIENTED_EDGE('',*,*,#47955,.F.);
#68597=ORIENTED_EDGE('',*,*,#50850,.F.);
#68598=ORIENTED_EDGE('',*,*,#48957,.F.);
#68599=ORIENTED_EDGE('',*,*,#50849,.T.);
#68600=ORIENTED_EDGE('',*,*,#48952,.F.);
#68601=ORIENTED_EDGE('',*,*,#50851,.F.);
#68602=ORIENTED_EDGE('',*,*,#46353,.F.);
#68603=ORIENTED_EDGE('',*,*,#47950,.F.);
#68604=ORIENTED_EDGE('',*,*,#47946,.T.);
#68605=ORIENTED_EDGE('',*,*,#50852,.F.);
#68606=ORIENTED_EDGE('',*,*,#48958,.F.);
#68607=ORIENTED_EDGE('',*,*,#50850,.T.);
#68608=ORIENTED_EDGE('',*,*,#50851,.T.);
#68609=ORIENTED_EDGE('',*,*,#50216,.F.);
#68610=ORIENTED_EDGE('',*,*,#50853,.F.);
#68611=ORIENTED_EDGE('',*,*,#46354,.F.);
#68612=ORIENTED_EDGE('',*,*,#50852,.T.);
#68613=ORIENTED_EDGE('',*,*,#47945,.F.);
#68614=ORIENTED_EDGE('',*,*,#50854,.F.);
#68615=ORIENTED_EDGE('',*,*,#48959,.F.);
#68616=ORIENTED_EDGE('',*,*,#50853,.T.);
#68617=ORIENTED_EDGE('',*,*,#48954,.F.);
#68618=ORIENTED_EDGE('',*,*,#50855,.F.);
#68619=ORIENTED_EDGE('',*,*,#46355,.F.);
#68620=ORIENTED_EDGE('',*,*,#50854,.T.);
#68621=ORIENTED_EDGE('',*,*,#47957,.F.);
#68622=ORIENTED_EDGE('',*,*,#50856,.F.);
#68623=ORIENTED_EDGE('',*,*,#48960,.F.);
#68624=ORIENTED_EDGE('',*,*,#50855,.T.);
#68625=ORIENTED_EDGE('',*,*,#48953,.F.);
#68626=ORIENTED_EDGE('',*,*,#50857,.F.);
#68627=ORIENTED_EDGE('',*,*,#47953,.F.);
#68628=ORIENTED_EDGE('',*,*,#50856,.T.);
#68629=ORIENTED_EDGE('',*,*,#47941,.F.);
#68630=ORIENTED_EDGE('',*,*,#50858,.F.);
#68631=ORIENTED_EDGE('',*,*,#48961,.F.);
#68632=ORIENTED_EDGE('',*,*,#50857,.T.);
#68633=ORIENTED_EDGE('',*,*,#48964,.F.);
#68634=ORIENTED_EDGE('',*,*,#50859,.F.);
#68635=ORIENTED_EDGE('',*,*,#47932,.F.);
#68636=ORIENTED_EDGE('',*,*,#50858,.T.);
#68637=ORIENTED_EDGE('',*,*,#47959,.F.);
#68638=ORIENTED_EDGE('',*,*,#50860,.F.);
#68639=ORIENTED_EDGE('',*,*,#48962,.F.);
#68640=ORIENTED_EDGE('',*,*,#50859,.T.);
#68641=ORIENTED_EDGE('',*,*,#48963,.F.);
#68642=ORIENTED_EDGE('',*,*,#50860,.T.);
#68643=ORIENTED_EDGE('',*,*,#47937,.F.);
#68644=ORIENTED_EDGE('',*,*,#47933,.T.);
#68645=ORIENTED_EDGE('',*,*,#50861,.F.);
#68646=ORIENTED_EDGE('',*,*,#49003,.F.);
#68647=ORIENTED_EDGE('',*,*,#50862,.F.);
#68648=ORIENTED_EDGE('',*,*,#47889,.F.);
#68649=ORIENTED_EDGE('',*,*,#50862,.T.);
#68650=ORIENTED_EDGE('',*,*,#49002,.F.);
#68651=ORIENTED_EDGE('',*,*,#50863,.F.);
#68652=ORIENTED_EDGE('',*,*,#47898,.F.);
#68653=ORIENTED_EDGE('',*,*,#47888,.T.);
#68654=ORIENTED_EDGE('',*,*,#47892,.F.);
#68655=ORIENTED_EDGE('',*,*,#50864,.F.);
#68656=ORIENTED_EDGE('',*,*,#49004,.F.);
#68657=ORIENTED_EDGE('',*,*,#50861,.T.);
#68658=ORIENTED_EDGE('',*,*,#50863,.T.);
#68659=ORIENTED_EDGE('',*,*,#49001,.F.);
#68660=ORIENTED_EDGE('',*,*,#50865,.F.);
#68661=ORIENTED_EDGE('',*,*,#47883,.F.);
#68662=ORIENTED_EDGE('',*,*,#50864,.T.);
#68663=ORIENTED_EDGE('',*,*,#47896,.F.);
#68664=ORIENTED_EDGE('',*,*,#50866,.F.);
#68665=ORIENTED_EDGE('',*,*,#48993,.F.);
#68666=ORIENTED_EDGE('',*,*,#50865,.T.);
#68667=ORIENTED_EDGE('',*,*,#49000,.F.);
#68668=ORIENTED_EDGE('',*,*,#50867,.F.);
#68669=ORIENTED_EDGE('',*,*,#47900,.F.);
#68670=ORIENTED_EDGE('',*,*,#50866,.T.);
#68671=ORIENTED_EDGE('',*,*,#46027,.F.);
#68672=ORIENTED_EDGE('',*,*,#50868,.F.);
#68673=ORIENTED_EDGE('',*,*,#48994,.F.);
#68674=ORIENTED_EDGE('',*,*,#50867,.T.);
#68675=ORIENTED_EDGE('',*,*,#48999,.F.);
#68676=ORIENTED_EDGE('',*,*,#50869,.F.);
#68677=ORIENTED_EDGE('',*,*,#47875,.T.);
#68678=ORIENTED_EDGE('',*,*,#47879,.F.);
#68679=ORIENTED_EDGE('',*,*,#50868,.T.);
#68680=ORIENTED_EDGE('',*,*,#46026,.F.);
#68681=ORIENTED_EDGE('',*,*,#50870,.F.);
#68682=ORIENTED_EDGE('',*,*,#50217,.F.);
#68683=ORIENTED_EDGE('',*,*,#50869,.T.);
#68684=ORIENTED_EDGE('',*,*,#48998,.F.);
#68685=ORIENTED_EDGE('',*,*,#50871,.F.);
#68686=ORIENTED_EDGE('',*,*,#47876,.F.);
#68687=ORIENTED_EDGE('',*,*,#50870,.T.);
#68688=ORIENTED_EDGE('',*,*,#46025,.F.);
#68689=ORIENTED_EDGE('',*,*,#50872,.F.);
#68690=ORIENTED_EDGE('',*,*,#48978,.F.);
#68691=ORIENTED_EDGE('',*,*,#50871,.T.);
#68692=ORIENTED_EDGE('',*,*,#48997,.F.);
#68693=ORIENTED_EDGE('',*,*,#50873,.F.);
#68694=ORIENTED_EDGE('',*,*,#47894,.F.);
#68695=ORIENTED_EDGE('',*,*,#50872,.T.);
#68696=ORIENTED_EDGE('',*,*,#46024,.F.);
#68697=ORIENTED_EDGE('',*,*,#50874,.F.);
#68698=ORIENTED_EDGE('',*,*,#50219,.F.);
#68699=ORIENTED_EDGE('',*,*,#50873,.T.);
#68700=ORIENTED_EDGE('',*,*,#48996,.F.);
#68701=ORIENTED_EDGE('',*,*,#50875,.F.);
#68702=ORIENTED_EDGE('',*,*,#46345,.F.);
#68703=ORIENTED_EDGE('',*,*,#50874,.T.);
#68704=ORIENTED_EDGE('',*,*,#46023,.F.);
#68705=ORIENTED_EDGE('',*,*,#50876,.F.);
#68706=ORIENTED_EDGE('',*,*,#48984,.F.);
#68707=ORIENTED_EDGE('',*,*,#50875,.T.);
#68708=ORIENTED_EDGE('',*,*,#50218,.F.);
#68709=ORIENTED_EDGE('',*,*,#50877,.F.);
#68710=ORIENTED_EDGE('',*,*,#46346,.F.);
#68711=ORIENTED_EDGE('',*,*,#50876,.T.);
#68712=ORIENTED_EDGE('',*,*,#47925,.F.);
#68713=ORIENTED_EDGE('',*,*,#50878,.F.);
#68714=ORIENTED_EDGE('',*,*,#48985,.F.);
#68715=ORIENTED_EDGE('',*,*,#50877,.T.);
#68716=ORIENTED_EDGE('',*,*,#48980,.F.);
#68717=ORIENTED_EDGE('',*,*,#50879,.F.);
#68718=ORIENTED_EDGE('',*,*,#46347,.F.);
#68719=ORIENTED_EDGE('',*,*,#47920,.F.);
#68720=ORIENTED_EDGE('',*,*,#47916,.T.);
#68721=ORIENTED_EDGE('',*,*,#50880,.F.);
#68722=ORIENTED_EDGE('',*,*,#48986,.F.);
#68723=ORIENTED_EDGE('',*,*,#50878,.T.);
#68724=ORIENTED_EDGE('',*,*,#50879,.T.);
#68725=ORIENTED_EDGE('',*,*,#50220,.F.);
#68726=ORIENTED_EDGE('',*,*,#50881,.F.);
#68727=ORIENTED_EDGE('',*,*,#46348,.F.);
#68728=ORIENTED_EDGE('',*,*,#50880,.T.);
#68729=ORIENTED_EDGE('',*,*,#47915,.F.);
#68730=ORIENTED_EDGE('',*,*,#50882,.F.);
#68731=ORIENTED_EDGE('',*,*,#48987,.F.);
#68732=ORIENTED_EDGE('',*,*,#50881,.T.);
#68733=ORIENTED_EDGE('',*,*,#48982,.F.);
#68734=ORIENTED_EDGE('',*,*,#50883,.F.);
#68735=ORIENTED_EDGE('',*,*,#46349,.F.);
#68736=ORIENTED_EDGE('',*,*,#50882,.T.);
#68737=ORIENTED_EDGE('',*,*,#47927,.F.);
#68738=ORIENTED_EDGE('',*,*,#50884,.F.);
#68739=ORIENTED_EDGE('',*,*,#48988,.F.);
#68740=ORIENTED_EDGE('',*,*,#50883,.T.);
#68741=ORIENTED_EDGE('',*,*,#48981,.F.);
#68742=ORIENTED_EDGE('',*,*,#50885,.F.);
#68743=ORIENTED_EDGE('',*,*,#47923,.F.);
#68744=ORIENTED_EDGE('',*,*,#50884,.T.);
#68745=ORIENTED_EDGE('',*,*,#47911,.F.);
#68746=ORIENTED_EDGE('',*,*,#50886,.F.);
#68747=ORIENTED_EDGE('',*,*,#48989,.F.);
#68748=ORIENTED_EDGE('',*,*,#50885,.T.);
#68749=ORIENTED_EDGE('',*,*,#48992,.F.);
#68750=ORIENTED_EDGE('',*,*,#50887,.F.);
#68751=ORIENTED_EDGE('',*,*,#47902,.F.);
#68752=ORIENTED_EDGE('',*,*,#50886,.T.);
#68753=ORIENTED_EDGE('',*,*,#47929,.F.);
#68754=ORIENTED_EDGE('',*,*,#50888,.F.);
#68755=ORIENTED_EDGE('',*,*,#48990,.F.);
#68756=ORIENTED_EDGE('',*,*,#50887,.T.);
#68757=ORIENTED_EDGE('',*,*,#48991,.F.);
#68758=ORIENTED_EDGE('',*,*,#50888,.T.);
#68759=ORIENTED_EDGE('',*,*,#47907,.F.);
#68760=ORIENTED_EDGE('',*,*,#47903,.T.);
#68761=ORIENTED_EDGE('',*,*,#50889,.F.);
#68762=ORIENTED_EDGE('',*,*,#49031,.F.);
#68763=ORIENTED_EDGE('',*,*,#50890,.F.);
#68764=ORIENTED_EDGE('',*,*,#47859,.F.);
#68765=ORIENTED_EDGE('',*,*,#50890,.T.);
#68766=ORIENTED_EDGE('',*,*,#49030,.F.);
#68767=ORIENTED_EDGE('',*,*,#50891,.F.);
#68768=ORIENTED_EDGE('',*,*,#47868,.F.);
#68769=ORIENTED_EDGE('',*,*,#47858,.T.);
#68770=ORIENTED_EDGE('',*,*,#47862,.F.);
#68771=ORIENTED_EDGE('',*,*,#50892,.F.);
#68772=ORIENTED_EDGE('',*,*,#49032,.F.);
#68773=ORIENTED_EDGE('',*,*,#50889,.T.);
#68774=ORIENTED_EDGE('',*,*,#50891,.T.);
#68775=ORIENTED_EDGE('',*,*,#49029,.F.);
#68776=ORIENTED_EDGE('',*,*,#50893,.F.);
#68777=ORIENTED_EDGE('',*,*,#47853,.F.);
#68778=ORIENTED_EDGE('',*,*,#50892,.T.);
#68779=ORIENTED_EDGE('',*,*,#47866,.F.);
#68780=ORIENTED_EDGE('',*,*,#50894,.F.);
#68781=ORIENTED_EDGE('',*,*,#49021,.F.);
#68782=ORIENTED_EDGE('',*,*,#50893,.T.);
#68783=ORIENTED_EDGE('',*,*,#49028,.F.);
#68784=ORIENTED_EDGE('',*,*,#50895,.F.);
#68785=ORIENTED_EDGE('',*,*,#47870,.F.);
#68786=ORIENTED_EDGE('',*,*,#50894,.T.);
#68787=ORIENTED_EDGE('',*,*,#46033,.F.);
#68788=ORIENTED_EDGE('',*,*,#50896,.F.);
#68789=ORIENTED_EDGE('',*,*,#49022,.F.);
#68790=ORIENTED_EDGE('',*,*,#50895,.T.);
#68791=ORIENTED_EDGE('',*,*,#49027,.F.);
#68792=ORIENTED_EDGE('',*,*,#50897,.F.);
#68793=ORIENTED_EDGE('',*,*,#47845,.T.);
#68794=ORIENTED_EDGE('',*,*,#47849,.F.);
#68795=ORIENTED_EDGE('',*,*,#50896,.T.);
#68796=ORIENTED_EDGE('',*,*,#46032,.F.);
#68797=ORIENTED_EDGE('',*,*,#50898,.F.);
#68798=ORIENTED_EDGE('',*,*,#50221,.F.);
#68799=ORIENTED_EDGE('',*,*,#50897,.T.);
#68800=ORIENTED_EDGE('',*,*,#49026,.F.);
#68801=ORIENTED_EDGE('',*,*,#50899,.F.);
#68802=ORIENTED_EDGE('',*,*,#47846,.F.);
#68803=ORIENTED_EDGE('',*,*,#50898,.T.);
#68804=ORIENTED_EDGE('',*,*,#46031,.F.);
#68805=ORIENTED_EDGE('',*,*,#50900,.F.);
#68806=ORIENTED_EDGE('',*,*,#49006,.F.);
#68807=ORIENTED_EDGE('',*,*,#50899,.T.);
#68808=ORIENTED_EDGE('',*,*,#49025,.F.);
#68809=ORIENTED_EDGE('',*,*,#50901,.F.);
#68810=ORIENTED_EDGE('',*,*,#47864,.F.);
#68811=ORIENTED_EDGE('',*,*,#50900,.T.);
#68812=ORIENTED_EDGE('',*,*,#46030,.F.);
#68813=ORIENTED_EDGE('',*,*,#50902,.F.);
#68814=ORIENTED_EDGE('',*,*,#50223,.F.);
#68815=ORIENTED_EDGE('',*,*,#50901,.T.);
#68816=ORIENTED_EDGE('',*,*,#49024,.F.);
#68817=ORIENTED_EDGE('',*,*,#50903,.F.);
#68818=ORIENTED_EDGE('',*,*,#46339,.F.);
#68819=ORIENTED_EDGE('',*,*,#50902,.T.);
#68820=ORIENTED_EDGE('',*,*,#46029,.F.);
#68821=ORIENTED_EDGE('',*,*,#50904,.F.);
#68822=ORIENTED_EDGE('',*,*,#49012,.F.);
#68823=ORIENTED_EDGE('',*,*,#50903,.T.);
#68824=ORIENTED_EDGE('',*,*,#50222,.F.);
#68825=ORIENTED_EDGE('',*,*,#50905,.F.);
#68826=ORIENTED_EDGE('',*,*,#46340,.F.);
#68827=ORIENTED_EDGE('',*,*,#50904,.T.);
#68828=ORIENTED_EDGE('',*,*,#47895,.F.);
#68829=ORIENTED_EDGE('',*,*,#50906,.F.);
#68830=ORIENTED_EDGE('',*,*,#49013,.F.);
#68831=ORIENTED_EDGE('',*,*,#50905,.T.);
#68832=ORIENTED_EDGE('',*,*,#49008,.F.);
#68833=ORIENTED_EDGE('',*,*,#50907,.F.);
#68834=ORIENTED_EDGE('',*,*,#46341,.F.);
#68835=ORIENTED_EDGE('',*,*,#47890,.F.);
#68836=ORIENTED_EDGE('',*,*,#47886,.T.);
#68837=ORIENTED_EDGE('',*,*,#50908,.F.);
#68838=ORIENTED_EDGE('',*,*,#49014,.F.);
#68839=ORIENTED_EDGE('',*,*,#50906,.T.);
#68840=ORIENTED_EDGE('',*,*,#50907,.T.);
#68841=ORIENTED_EDGE('',*,*,#50224,.F.);
#68842=ORIENTED_EDGE('',*,*,#50909,.F.);
#68843=ORIENTED_EDGE('',*,*,#46342,.F.);
#68844=ORIENTED_EDGE('',*,*,#50908,.T.);
#68845=ORIENTED_EDGE('',*,*,#47885,.F.);
#68846=ORIENTED_EDGE('',*,*,#50910,.F.);
#68847=ORIENTED_EDGE('',*,*,#49015,.F.);
#68848=ORIENTED_EDGE('',*,*,#50909,.T.);
#68849=ORIENTED_EDGE('',*,*,#49010,.F.);
#68850=ORIENTED_EDGE('',*,*,#50911,.F.);
#68851=ORIENTED_EDGE('',*,*,#46343,.F.);
#68852=ORIENTED_EDGE('',*,*,#50910,.T.);
#68853=ORIENTED_EDGE('',*,*,#47897,.F.);
#68854=ORIENTED_EDGE('',*,*,#50912,.F.);
#68855=ORIENTED_EDGE('',*,*,#49016,.F.);
#68856=ORIENTED_EDGE('',*,*,#50911,.T.);
#68857=ORIENTED_EDGE('',*,*,#49009,.F.);
#68858=ORIENTED_EDGE('',*,*,#50913,.F.);
#68859=ORIENTED_EDGE('',*,*,#47893,.F.);
#68860=ORIENTED_EDGE('',*,*,#50912,.T.);
#68861=ORIENTED_EDGE('',*,*,#47881,.F.);
#68862=ORIENTED_EDGE('',*,*,#50914,.F.);
#68863=ORIENTED_EDGE('',*,*,#49017,.F.);
#68864=ORIENTED_EDGE('',*,*,#50913,.T.);
#68865=ORIENTED_EDGE('',*,*,#49020,.F.);
#68866=ORIENTED_EDGE('',*,*,#50915,.F.);
#68867=ORIENTED_EDGE('',*,*,#47872,.F.);
#68868=ORIENTED_EDGE('',*,*,#50914,.T.);
#68869=ORIENTED_EDGE('',*,*,#47899,.F.);
#68870=ORIENTED_EDGE('',*,*,#50916,.F.);
#68871=ORIENTED_EDGE('',*,*,#49018,.F.);
#68872=ORIENTED_EDGE('',*,*,#50915,.T.);
#68873=ORIENTED_EDGE('',*,*,#49019,.F.);
#68874=ORIENTED_EDGE('',*,*,#50916,.T.);
#68875=ORIENTED_EDGE('',*,*,#47877,.F.);
#68876=ORIENTED_EDGE('',*,*,#47873,.T.);
#68877=ORIENTED_EDGE('',*,*,#50917,.F.);
#68878=ORIENTED_EDGE('',*,*,#49059,.F.);
#68879=ORIENTED_EDGE('',*,*,#50918,.F.);
#68880=ORIENTED_EDGE('',*,*,#47829,.F.);
#68881=ORIENTED_EDGE('',*,*,#50918,.T.);
#68882=ORIENTED_EDGE('',*,*,#49058,.F.);
#68883=ORIENTED_EDGE('',*,*,#50919,.F.);
#68884=ORIENTED_EDGE('',*,*,#47838,.F.);
#68885=ORIENTED_EDGE('',*,*,#47828,.T.);
#68886=ORIENTED_EDGE('',*,*,#47832,.F.);
#68887=ORIENTED_EDGE('',*,*,#50920,.F.);
#68888=ORIENTED_EDGE('',*,*,#49060,.F.);
#68889=ORIENTED_EDGE('',*,*,#50917,.T.);
#68890=ORIENTED_EDGE('',*,*,#50919,.T.);
#68891=ORIENTED_EDGE('',*,*,#49057,.F.);
#68892=ORIENTED_EDGE('',*,*,#50921,.F.);
#68893=ORIENTED_EDGE('',*,*,#47823,.F.);
#68894=ORIENTED_EDGE('',*,*,#50920,.T.);
#68895=ORIENTED_EDGE('',*,*,#47836,.F.);
#68896=ORIENTED_EDGE('',*,*,#50922,.F.);
#68897=ORIENTED_EDGE('',*,*,#49049,.F.);
#68898=ORIENTED_EDGE('',*,*,#50921,.T.);
#68899=ORIENTED_EDGE('',*,*,#49056,.F.);
#68900=ORIENTED_EDGE('',*,*,#50923,.F.);
#68901=ORIENTED_EDGE('',*,*,#47840,.F.);
#68902=ORIENTED_EDGE('',*,*,#50922,.T.);
#68903=ORIENTED_EDGE('',*,*,#46039,.F.);
#68904=ORIENTED_EDGE('',*,*,#50924,.F.);
#68905=ORIENTED_EDGE('',*,*,#49050,.F.);
#68906=ORIENTED_EDGE('',*,*,#50923,.T.);
#68907=ORIENTED_EDGE('',*,*,#49055,.F.);
#68908=ORIENTED_EDGE('',*,*,#50925,.F.);
#68909=ORIENTED_EDGE('',*,*,#47815,.T.);
#68910=ORIENTED_EDGE('',*,*,#47819,.F.);
#68911=ORIENTED_EDGE('',*,*,#50924,.T.);
#68912=ORIENTED_EDGE('',*,*,#46038,.F.);
#68913=ORIENTED_EDGE('',*,*,#50926,.F.);
#68914=ORIENTED_EDGE('',*,*,#50225,.F.);
#68915=ORIENTED_EDGE('',*,*,#50925,.T.);
#68916=ORIENTED_EDGE('',*,*,#49054,.F.);
#68917=ORIENTED_EDGE('',*,*,#50927,.F.);
#68918=ORIENTED_EDGE('',*,*,#47816,.F.);
#68919=ORIENTED_EDGE('',*,*,#50926,.T.);
#68920=ORIENTED_EDGE('',*,*,#46037,.F.);
#68921=ORIENTED_EDGE('',*,*,#50928,.F.);
#68922=ORIENTED_EDGE('',*,*,#49034,.F.);
#68923=ORIENTED_EDGE('',*,*,#50927,.T.);
#68924=ORIENTED_EDGE('',*,*,#49053,.F.);
#68925=ORIENTED_EDGE('',*,*,#50929,.F.);
#68926=ORIENTED_EDGE('',*,*,#47834,.F.);
#68927=ORIENTED_EDGE('',*,*,#50928,.T.);
#68928=ORIENTED_EDGE('',*,*,#46036,.F.);
#68929=ORIENTED_EDGE('',*,*,#50930,.F.);
#68930=ORIENTED_EDGE('',*,*,#50227,.F.);
#68931=ORIENTED_EDGE('',*,*,#50929,.T.);
#68932=ORIENTED_EDGE('',*,*,#49052,.F.);
#68933=ORIENTED_EDGE('',*,*,#50931,.F.);
#68934=ORIENTED_EDGE('',*,*,#46333,.F.);
#68935=ORIENTED_EDGE('',*,*,#50930,.T.);
#68936=ORIENTED_EDGE('',*,*,#46035,.F.);
#68937=ORIENTED_EDGE('',*,*,#50932,.F.);
#68938=ORIENTED_EDGE('',*,*,#49040,.F.);
#68939=ORIENTED_EDGE('',*,*,#50931,.T.);
#68940=ORIENTED_EDGE('',*,*,#50226,.F.);
#68941=ORIENTED_EDGE('',*,*,#50933,.F.);
#68942=ORIENTED_EDGE('',*,*,#46334,.F.);
#68943=ORIENTED_EDGE('',*,*,#50932,.T.);
#68944=ORIENTED_EDGE('',*,*,#47865,.F.);
#68945=ORIENTED_EDGE('',*,*,#50934,.F.);
#68946=ORIENTED_EDGE('',*,*,#49041,.F.);
#68947=ORIENTED_EDGE('',*,*,#50933,.T.);
#68948=ORIENTED_EDGE('',*,*,#49036,.F.);
#68949=ORIENTED_EDGE('',*,*,#50935,.F.);
#68950=ORIENTED_EDGE('',*,*,#46335,.F.);
#68951=ORIENTED_EDGE('',*,*,#47860,.F.);
#68952=ORIENTED_EDGE('',*,*,#47856,.T.);
#68953=ORIENTED_EDGE('',*,*,#50936,.F.);
#68954=ORIENTED_EDGE('',*,*,#49042,.F.);
#68955=ORIENTED_EDGE('',*,*,#50934,.T.);
#68956=ORIENTED_EDGE('',*,*,#50935,.T.);
#68957=ORIENTED_EDGE('',*,*,#50228,.F.);
#68958=ORIENTED_EDGE('',*,*,#50937,.F.);
#68959=ORIENTED_EDGE('',*,*,#46336,.F.);
#68960=ORIENTED_EDGE('',*,*,#50936,.T.);
#68961=ORIENTED_EDGE('',*,*,#47855,.F.);
#68962=ORIENTED_EDGE('',*,*,#50938,.F.);
#68963=ORIENTED_EDGE('',*,*,#49043,.F.);
#68964=ORIENTED_EDGE('',*,*,#50937,.T.);
#68965=ORIENTED_EDGE('',*,*,#49038,.F.);
#68966=ORIENTED_EDGE('',*,*,#50939,.F.);
#68967=ORIENTED_EDGE('',*,*,#46337,.F.);
#68968=ORIENTED_EDGE('',*,*,#50938,.T.);
#68969=ORIENTED_EDGE('',*,*,#47867,.F.);
#68970=ORIENTED_EDGE('',*,*,#50940,.F.);
#68971=ORIENTED_EDGE('',*,*,#49044,.F.);
#68972=ORIENTED_EDGE('',*,*,#50939,.T.);
#68973=ORIENTED_EDGE('',*,*,#49037,.F.);
#68974=ORIENTED_EDGE('',*,*,#50941,.F.);
#68975=ORIENTED_EDGE('',*,*,#47863,.F.);
#68976=ORIENTED_EDGE('',*,*,#50940,.T.);
#68977=ORIENTED_EDGE('',*,*,#47851,.F.);
#68978=ORIENTED_EDGE('',*,*,#50942,.F.);
#68979=ORIENTED_EDGE('',*,*,#49045,.F.);
#68980=ORIENTED_EDGE('',*,*,#50941,.T.);
#68981=ORIENTED_EDGE('',*,*,#49048,.F.);
#68982=ORIENTED_EDGE('',*,*,#50943,.F.);
#68983=ORIENTED_EDGE('',*,*,#47842,.F.);
#68984=ORIENTED_EDGE('',*,*,#50942,.T.);
#68985=ORIENTED_EDGE('',*,*,#47869,.F.);
#68986=ORIENTED_EDGE('',*,*,#50944,.F.);
#68987=ORIENTED_EDGE('',*,*,#49046,.F.);
#68988=ORIENTED_EDGE('',*,*,#50943,.T.);
#68989=ORIENTED_EDGE('',*,*,#49047,.F.);
#68990=ORIENTED_EDGE('',*,*,#50944,.T.);
#68991=ORIENTED_EDGE('',*,*,#47847,.F.);
#68992=ORIENTED_EDGE('',*,*,#47843,.T.);
#68993=ORIENTED_EDGE('',*,*,#50945,.F.);
#68994=ORIENTED_EDGE('',*,*,#49087,.F.);
#68995=ORIENTED_EDGE('',*,*,#50946,.F.);
#68996=ORIENTED_EDGE('',*,*,#47799,.F.);
#68997=ORIENTED_EDGE('',*,*,#50946,.T.);
#68998=ORIENTED_EDGE('',*,*,#49086,.F.);
#68999=ORIENTED_EDGE('',*,*,#50947,.F.);
#69000=ORIENTED_EDGE('',*,*,#47808,.F.);
#69001=ORIENTED_EDGE('',*,*,#47798,.T.);
#69002=ORIENTED_EDGE('',*,*,#47802,.F.);
#69003=ORIENTED_EDGE('',*,*,#50948,.F.);
#69004=ORIENTED_EDGE('',*,*,#49088,.F.);
#69005=ORIENTED_EDGE('',*,*,#50945,.T.);
#69006=ORIENTED_EDGE('',*,*,#50947,.T.);
#69007=ORIENTED_EDGE('',*,*,#49085,.F.);
#69008=ORIENTED_EDGE('',*,*,#50949,.F.);
#69009=ORIENTED_EDGE('',*,*,#47793,.F.);
#69010=ORIENTED_EDGE('',*,*,#50948,.T.);
#69011=ORIENTED_EDGE('',*,*,#47806,.F.);
#69012=ORIENTED_EDGE('',*,*,#50950,.F.);
#69013=ORIENTED_EDGE('',*,*,#49077,.F.);
#69014=ORIENTED_EDGE('',*,*,#50949,.T.);
#69015=ORIENTED_EDGE('',*,*,#49084,.F.);
#69016=ORIENTED_EDGE('',*,*,#50951,.F.);
#69017=ORIENTED_EDGE('',*,*,#47810,.F.);
#69018=ORIENTED_EDGE('',*,*,#50950,.T.);
#69019=ORIENTED_EDGE('',*,*,#46045,.F.);
#69020=ORIENTED_EDGE('',*,*,#50952,.F.);
#69021=ORIENTED_EDGE('',*,*,#49078,.F.);
#69022=ORIENTED_EDGE('',*,*,#50951,.T.);
#69023=ORIENTED_EDGE('',*,*,#49083,.F.);
#69024=ORIENTED_EDGE('',*,*,#50953,.F.);
#69025=ORIENTED_EDGE('',*,*,#47785,.T.);
#69026=ORIENTED_EDGE('',*,*,#47789,.F.);
#69027=ORIENTED_EDGE('',*,*,#50952,.T.);
#69028=ORIENTED_EDGE('',*,*,#46044,.F.);
#69029=ORIENTED_EDGE('',*,*,#50954,.F.);
#69030=ORIENTED_EDGE('',*,*,#50229,.F.);
#69031=ORIENTED_EDGE('',*,*,#50953,.T.);
#69032=ORIENTED_EDGE('',*,*,#49082,.F.);
#69033=ORIENTED_EDGE('',*,*,#50955,.F.);
#69034=ORIENTED_EDGE('',*,*,#47786,.F.);
#69035=ORIENTED_EDGE('',*,*,#50954,.T.);
#69036=ORIENTED_EDGE('',*,*,#46043,.F.);
#69037=ORIENTED_EDGE('',*,*,#50956,.F.);
#69038=ORIENTED_EDGE('',*,*,#49062,.F.);
#69039=ORIENTED_EDGE('',*,*,#50955,.T.);
#69040=ORIENTED_EDGE('',*,*,#49081,.F.);
#69041=ORIENTED_EDGE('',*,*,#50957,.F.);
#69042=ORIENTED_EDGE('',*,*,#47804,.F.);
#69043=ORIENTED_EDGE('',*,*,#50956,.T.);
#69044=ORIENTED_EDGE('',*,*,#46042,.F.);
#69045=ORIENTED_EDGE('',*,*,#50958,.F.);
#69046=ORIENTED_EDGE('',*,*,#50231,.F.);
#69047=ORIENTED_EDGE('',*,*,#50957,.T.);
#69048=ORIENTED_EDGE('',*,*,#49080,.F.);
#69049=ORIENTED_EDGE('',*,*,#50959,.F.);
#69050=ORIENTED_EDGE('',*,*,#46327,.F.);
#69051=ORIENTED_EDGE('',*,*,#50958,.T.);
#69052=ORIENTED_EDGE('',*,*,#46041,.F.);
#69053=ORIENTED_EDGE('',*,*,#50960,.F.);
#69054=ORIENTED_EDGE('',*,*,#49068,.F.);
#69055=ORIENTED_EDGE('',*,*,#50959,.T.);
#69056=ORIENTED_EDGE('',*,*,#50230,.F.);
#69057=ORIENTED_EDGE('',*,*,#50961,.F.);
#69058=ORIENTED_EDGE('',*,*,#46328,.F.);
#69059=ORIENTED_EDGE('',*,*,#50960,.T.);
#69060=ORIENTED_EDGE('',*,*,#47835,.F.);
#69061=ORIENTED_EDGE('',*,*,#50962,.F.);
#69062=ORIENTED_EDGE('',*,*,#49069,.F.);
#69063=ORIENTED_EDGE('',*,*,#50961,.T.);
#69064=ORIENTED_EDGE('',*,*,#49064,.F.);
#69065=ORIENTED_EDGE('',*,*,#50963,.F.);
#69066=ORIENTED_EDGE('',*,*,#46329,.F.);
#69067=ORIENTED_EDGE('',*,*,#47830,.F.);
#69068=ORIENTED_EDGE('',*,*,#47826,.T.);
#69069=ORIENTED_EDGE('',*,*,#50964,.F.);
#69070=ORIENTED_EDGE('',*,*,#49070,.F.);
#69071=ORIENTED_EDGE('',*,*,#50962,.T.);
#69072=ORIENTED_EDGE('',*,*,#50963,.T.);
#69073=ORIENTED_EDGE('',*,*,#50232,.F.);
#69074=ORIENTED_EDGE('',*,*,#50965,.F.);
#69075=ORIENTED_EDGE('',*,*,#46330,.F.);
#69076=ORIENTED_EDGE('',*,*,#50964,.T.);
#69077=ORIENTED_EDGE('',*,*,#47825,.F.);
#69078=ORIENTED_EDGE('',*,*,#50966,.F.);
#69079=ORIENTED_EDGE('',*,*,#49071,.F.);
#69080=ORIENTED_EDGE('',*,*,#50965,.T.);
#69081=ORIENTED_EDGE('',*,*,#49066,.F.);
#69082=ORIENTED_EDGE('',*,*,#50967,.F.);
#69083=ORIENTED_EDGE('',*,*,#46331,.F.);
#69084=ORIENTED_EDGE('',*,*,#50966,.T.);
#69085=ORIENTED_EDGE('',*,*,#47837,.F.);
#69086=ORIENTED_EDGE('',*,*,#50968,.F.);
#69087=ORIENTED_EDGE('',*,*,#49072,.F.);
#69088=ORIENTED_EDGE('',*,*,#50967,.T.);
#69089=ORIENTED_EDGE('',*,*,#49065,.F.);
#69090=ORIENTED_EDGE('',*,*,#50969,.F.);
#69091=ORIENTED_EDGE('',*,*,#47833,.F.);
#69092=ORIENTED_EDGE('',*,*,#50968,.T.);
#69093=ORIENTED_EDGE('',*,*,#47821,.F.);
#69094=ORIENTED_EDGE('',*,*,#50970,.F.);
#69095=ORIENTED_EDGE('',*,*,#49073,.F.);
#69096=ORIENTED_EDGE('',*,*,#50969,.T.);
#69097=ORIENTED_EDGE('',*,*,#49076,.F.);
#69098=ORIENTED_EDGE('',*,*,#50971,.F.);
#69099=ORIENTED_EDGE('',*,*,#47812,.F.);
#69100=ORIENTED_EDGE('',*,*,#50970,.T.);
#69101=ORIENTED_EDGE('',*,*,#47839,.F.);
#69102=ORIENTED_EDGE('',*,*,#50972,.F.);
#69103=ORIENTED_EDGE('',*,*,#49074,.F.);
#69104=ORIENTED_EDGE('',*,*,#50971,.T.);
#69105=ORIENTED_EDGE('',*,*,#49075,.F.);
#69106=ORIENTED_EDGE('',*,*,#50972,.T.);
#69107=ORIENTED_EDGE('',*,*,#47817,.F.);
#69108=ORIENTED_EDGE('',*,*,#47813,.T.);
#69109=ORIENTED_EDGE('',*,*,#50973,.F.);
#69110=ORIENTED_EDGE('',*,*,#49115,.F.);
#69111=ORIENTED_EDGE('',*,*,#50974,.F.);
#69112=ORIENTED_EDGE('',*,*,#47769,.F.);
#69113=ORIENTED_EDGE('',*,*,#50974,.T.);
#69114=ORIENTED_EDGE('',*,*,#49114,.F.);
#69115=ORIENTED_EDGE('',*,*,#50975,.F.);
#69116=ORIENTED_EDGE('',*,*,#47778,.F.);
#69117=ORIENTED_EDGE('',*,*,#47768,.T.);
#69118=ORIENTED_EDGE('',*,*,#47772,.F.);
#69119=ORIENTED_EDGE('',*,*,#50976,.F.);
#69120=ORIENTED_EDGE('',*,*,#49116,.F.);
#69121=ORIENTED_EDGE('',*,*,#50973,.T.);
#69122=ORIENTED_EDGE('',*,*,#50975,.T.);
#69123=ORIENTED_EDGE('',*,*,#49113,.F.);
#69124=ORIENTED_EDGE('',*,*,#50977,.F.);
#69125=ORIENTED_EDGE('',*,*,#47763,.F.);
#69126=ORIENTED_EDGE('',*,*,#50976,.T.);
#69127=ORIENTED_EDGE('',*,*,#47776,.F.);
#69128=ORIENTED_EDGE('',*,*,#50978,.F.);
#69129=ORIENTED_EDGE('',*,*,#49105,.F.);
#69130=ORIENTED_EDGE('',*,*,#50977,.T.);
#69131=ORIENTED_EDGE('',*,*,#49112,.F.);
#69132=ORIENTED_EDGE('',*,*,#50979,.F.);
#69133=ORIENTED_EDGE('',*,*,#47780,.F.);
#69134=ORIENTED_EDGE('',*,*,#50978,.T.);
#69135=ORIENTED_EDGE('',*,*,#46051,.F.);
#69136=ORIENTED_EDGE('',*,*,#50980,.F.);
#69137=ORIENTED_EDGE('',*,*,#49106,.F.);
#69138=ORIENTED_EDGE('',*,*,#50979,.T.);
#69139=ORIENTED_EDGE('',*,*,#49111,.F.);
#69140=ORIENTED_EDGE('',*,*,#50981,.F.);
#69141=ORIENTED_EDGE('',*,*,#47755,.T.);
#69142=ORIENTED_EDGE('',*,*,#47759,.F.);
#69143=ORIENTED_EDGE('',*,*,#50980,.T.);
#69144=ORIENTED_EDGE('',*,*,#46050,.F.);
#69145=ORIENTED_EDGE('',*,*,#50982,.F.);
#69146=ORIENTED_EDGE('',*,*,#50233,.F.);
#69147=ORIENTED_EDGE('',*,*,#50981,.T.);
#69148=ORIENTED_EDGE('',*,*,#49110,.F.);
#69149=ORIENTED_EDGE('',*,*,#50983,.F.);
#69150=ORIENTED_EDGE('',*,*,#47756,.F.);
#69151=ORIENTED_EDGE('',*,*,#50982,.T.);
#69152=ORIENTED_EDGE('',*,*,#46049,.F.);
#69153=ORIENTED_EDGE('',*,*,#50984,.F.);
#69154=ORIENTED_EDGE('',*,*,#49090,.F.);
#69155=ORIENTED_EDGE('',*,*,#50983,.T.);
#69156=ORIENTED_EDGE('',*,*,#49109,.F.);
#69157=ORIENTED_EDGE('',*,*,#50985,.F.);
#69158=ORIENTED_EDGE('',*,*,#47774,.F.);
#69159=ORIENTED_EDGE('',*,*,#50984,.T.);
#69160=ORIENTED_EDGE('',*,*,#46048,.F.);
#69161=ORIENTED_EDGE('',*,*,#50986,.F.);
#69162=ORIENTED_EDGE('',*,*,#50235,.F.);
#69163=ORIENTED_EDGE('',*,*,#50985,.T.);
#69164=ORIENTED_EDGE('',*,*,#49108,.F.);
#69165=ORIENTED_EDGE('',*,*,#50987,.F.);
#69166=ORIENTED_EDGE('',*,*,#46321,.F.);
#69167=ORIENTED_EDGE('',*,*,#50986,.T.);
#69168=ORIENTED_EDGE('',*,*,#46047,.F.);
#69169=ORIENTED_EDGE('',*,*,#50988,.F.);
#69170=ORIENTED_EDGE('',*,*,#49096,.F.);
#69171=ORIENTED_EDGE('',*,*,#50987,.T.);
#69172=ORIENTED_EDGE('',*,*,#50234,.F.);
#69173=ORIENTED_EDGE('',*,*,#50989,.F.);
#69174=ORIENTED_EDGE('',*,*,#46322,.F.);
#69175=ORIENTED_EDGE('',*,*,#50988,.T.);
#69176=ORIENTED_EDGE('',*,*,#47805,.F.);
#69177=ORIENTED_EDGE('',*,*,#50990,.F.);
#69178=ORIENTED_EDGE('',*,*,#49097,.F.);
#69179=ORIENTED_EDGE('',*,*,#50989,.T.);
#69180=ORIENTED_EDGE('',*,*,#49092,.F.);
#69181=ORIENTED_EDGE('',*,*,#50991,.F.);
#69182=ORIENTED_EDGE('',*,*,#46323,.F.);
#69183=ORIENTED_EDGE('',*,*,#47800,.F.);
#69184=ORIENTED_EDGE('',*,*,#47796,.T.);
#69185=ORIENTED_EDGE('',*,*,#50992,.F.);
#69186=ORIENTED_EDGE('',*,*,#49098,.F.);
#69187=ORIENTED_EDGE('',*,*,#50990,.T.);
#69188=ORIENTED_EDGE('',*,*,#50991,.T.);
#69189=ORIENTED_EDGE('',*,*,#50236,.F.);
#69190=ORIENTED_EDGE('',*,*,#50993,.F.);
#69191=ORIENTED_EDGE('',*,*,#46324,.F.);
#69192=ORIENTED_EDGE('',*,*,#50992,.T.);
#69193=ORIENTED_EDGE('',*,*,#47795,.F.);
#69194=ORIENTED_EDGE('',*,*,#50994,.F.);
#69195=ORIENTED_EDGE('',*,*,#49099,.F.);
#69196=ORIENTED_EDGE('',*,*,#50993,.T.);
#69197=ORIENTED_EDGE('',*,*,#49094,.F.);
#69198=ORIENTED_EDGE('',*,*,#50995,.F.);
#69199=ORIENTED_EDGE('',*,*,#46325,.F.);
#69200=ORIENTED_EDGE('',*,*,#50994,.T.);
#69201=ORIENTED_EDGE('',*,*,#47807,.F.);
#69202=ORIENTED_EDGE('',*,*,#50996,.F.);
#69203=ORIENTED_EDGE('',*,*,#49100,.F.);
#69204=ORIENTED_EDGE('',*,*,#50995,.T.);
#69205=ORIENTED_EDGE('',*,*,#49093,.F.);
#69206=ORIENTED_EDGE('',*,*,#50997,.F.);
#69207=ORIENTED_EDGE('',*,*,#47803,.F.);
#69208=ORIENTED_EDGE('',*,*,#50996,.T.);
#69209=ORIENTED_EDGE('',*,*,#47791,.F.);
#69210=ORIENTED_EDGE('',*,*,#50998,.F.);
#69211=ORIENTED_EDGE('',*,*,#49101,.F.);
#69212=ORIENTED_EDGE('',*,*,#50997,.T.);
#69213=ORIENTED_EDGE('',*,*,#49104,.F.);
#69214=ORIENTED_EDGE('',*,*,#50999,.F.);
#69215=ORIENTED_EDGE('',*,*,#47782,.F.);
#69216=ORIENTED_EDGE('',*,*,#50998,.T.);
#69217=ORIENTED_EDGE('',*,*,#47809,.F.);
#69218=ORIENTED_EDGE('',*,*,#51000,.F.);
#69219=ORIENTED_EDGE('',*,*,#49102,.F.);
#69220=ORIENTED_EDGE('',*,*,#50999,.T.);
#69221=ORIENTED_EDGE('',*,*,#49103,.F.);
#69222=ORIENTED_EDGE('',*,*,#51000,.T.);
#69223=ORIENTED_EDGE('',*,*,#47787,.F.);
#69224=ORIENTED_EDGE('',*,*,#47783,.T.);
#69225=ORIENTED_EDGE('',*,*,#51001,.F.);
#69226=ORIENTED_EDGE('',*,*,#49143,.F.);
#69227=ORIENTED_EDGE('',*,*,#51002,.F.);
#69228=ORIENTED_EDGE('',*,*,#47739,.F.);
#69229=ORIENTED_EDGE('',*,*,#51002,.T.);
#69230=ORIENTED_EDGE('',*,*,#49142,.F.);
#69231=ORIENTED_EDGE('',*,*,#51003,.F.);
#69232=ORIENTED_EDGE('',*,*,#47748,.F.);
#69233=ORIENTED_EDGE('',*,*,#47738,.T.);
#69234=ORIENTED_EDGE('',*,*,#47742,.F.);
#69235=ORIENTED_EDGE('',*,*,#51004,.F.);
#69236=ORIENTED_EDGE('',*,*,#49144,.F.);
#69237=ORIENTED_EDGE('',*,*,#51001,.T.);
#69238=ORIENTED_EDGE('',*,*,#51003,.T.);
#69239=ORIENTED_EDGE('',*,*,#49141,.F.);
#69240=ORIENTED_EDGE('',*,*,#51005,.F.);
#69241=ORIENTED_EDGE('',*,*,#47733,.F.);
#69242=ORIENTED_EDGE('',*,*,#51004,.T.);
#69243=ORIENTED_EDGE('',*,*,#47746,.F.);
#69244=ORIENTED_EDGE('',*,*,#51006,.F.);
#69245=ORIENTED_EDGE('',*,*,#49133,.F.);
#69246=ORIENTED_EDGE('',*,*,#51005,.T.);
#69247=ORIENTED_EDGE('',*,*,#49140,.F.);
#69248=ORIENTED_EDGE('',*,*,#51007,.F.);
#69249=ORIENTED_EDGE('',*,*,#47750,.F.);
#69250=ORIENTED_EDGE('',*,*,#51006,.T.);
#69251=ORIENTED_EDGE('',*,*,#46057,.F.);
#69252=ORIENTED_EDGE('',*,*,#51008,.F.);
#69253=ORIENTED_EDGE('',*,*,#49134,.F.);
#69254=ORIENTED_EDGE('',*,*,#51007,.T.);
#69255=ORIENTED_EDGE('',*,*,#49139,.F.);
#69256=ORIENTED_EDGE('',*,*,#51009,.F.);
#69257=ORIENTED_EDGE('',*,*,#47725,.T.);
#69258=ORIENTED_EDGE('',*,*,#47729,.F.);
#69259=ORIENTED_EDGE('',*,*,#51008,.T.);
#69260=ORIENTED_EDGE('',*,*,#46056,.F.);
#69261=ORIENTED_EDGE('',*,*,#51010,.F.);
#69262=ORIENTED_EDGE('',*,*,#50237,.F.);
#69263=ORIENTED_EDGE('',*,*,#51009,.T.);
#69264=ORIENTED_EDGE('',*,*,#49138,.F.);
#69265=ORIENTED_EDGE('',*,*,#51011,.F.);
#69266=ORIENTED_EDGE('',*,*,#47726,.F.);
#69267=ORIENTED_EDGE('',*,*,#51010,.T.);
#69268=ORIENTED_EDGE('',*,*,#46055,.F.);
#69269=ORIENTED_EDGE('',*,*,#51012,.F.);
#69270=ORIENTED_EDGE('',*,*,#49118,.F.);
#69271=ORIENTED_EDGE('',*,*,#51011,.T.);
#69272=ORIENTED_EDGE('',*,*,#49137,.F.);
#69273=ORIENTED_EDGE('',*,*,#51013,.F.);
#69274=ORIENTED_EDGE('',*,*,#47744,.F.);
#69275=ORIENTED_EDGE('',*,*,#51012,.T.);
#69276=ORIENTED_EDGE('',*,*,#46054,.F.);
#69277=ORIENTED_EDGE('',*,*,#51014,.F.);
#69278=ORIENTED_EDGE('',*,*,#50239,.F.);
#69279=ORIENTED_EDGE('',*,*,#51013,.T.);
#69280=ORIENTED_EDGE('',*,*,#49136,.F.);
#69281=ORIENTED_EDGE('',*,*,#51015,.F.);
#69282=ORIENTED_EDGE('',*,*,#46315,.F.);
#69283=ORIENTED_EDGE('',*,*,#51014,.T.);
#69284=ORIENTED_EDGE('',*,*,#46053,.F.);
#69285=ORIENTED_EDGE('',*,*,#51016,.F.);
#69286=ORIENTED_EDGE('',*,*,#49124,.F.);
#69287=ORIENTED_EDGE('',*,*,#51015,.T.);
#69288=ORIENTED_EDGE('',*,*,#50238,.F.);
#69289=ORIENTED_EDGE('',*,*,#51017,.F.);
#69290=ORIENTED_EDGE('',*,*,#46316,.F.);
#69291=ORIENTED_EDGE('',*,*,#51016,.T.);
#69292=ORIENTED_EDGE('',*,*,#47775,.F.);
#69293=ORIENTED_EDGE('',*,*,#51018,.F.);
#69294=ORIENTED_EDGE('',*,*,#49125,.F.);
#69295=ORIENTED_EDGE('',*,*,#51017,.T.);
#69296=ORIENTED_EDGE('',*,*,#49120,.F.);
#69297=ORIENTED_EDGE('',*,*,#51019,.F.);
#69298=ORIENTED_EDGE('',*,*,#46317,.F.);
#69299=ORIENTED_EDGE('',*,*,#47770,.F.);
#69300=ORIENTED_EDGE('',*,*,#47766,.T.);
#69301=ORIENTED_EDGE('',*,*,#51020,.F.);
#69302=ORIENTED_EDGE('',*,*,#49126,.F.);
#69303=ORIENTED_EDGE('',*,*,#51018,.T.);
#69304=ORIENTED_EDGE('',*,*,#51019,.T.);
#69305=ORIENTED_EDGE('',*,*,#50240,.F.);
#69306=ORIENTED_EDGE('',*,*,#51021,.F.);
#69307=ORIENTED_EDGE('',*,*,#46318,.F.);
#69308=ORIENTED_EDGE('',*,*,#51020,.T.);
#69309=ORIENTED_EDGE('',*,*,#47765,.F.);
#69310=ORIENTED_EDGE('',*,*,#51022,.F.);
#69311=ORIENTED_EDGE('',*,*,#49127,.F.);
#69312=ORIENTED_EDGE('',*,*,#51021,.T.);
#69313=ORIENTED_EDGE('',*,*,#49122,.F.);
#69314=ORIENTED_EDGE('',*,*,#51023,.F.);
#69315=ORIENTED_EDGE('',*,*,#46319,.F.);
#69316=ORIENTED_EDGE('',*,*,#51022,.T.);
#69317=ORIENTED_EDGE('',*,*,#47777,.F.);
#69318=ORIENTED_EDGE('',*,*,#51024,.F.);
#69319=ORIENTED_EDGE('',*,*,#49128,.F.);
#69320=ORIENTED_EDGE('',*,*,#51023,.T.);
#69321=ORIENTED_EDGE('',*,*,#49121,.F.);
#69322=ORIENTED_EDGE('',*,*,#51025,.F.);
#69323=ORIENTED_EDGE('',*,*,#47773,.F.);
#69324=ORIENTED_EDGE('',*,*,#51024,.T.);
#69325=ORIENTED_EDGE('',*,*,#47761,.F.);
#69326=ORIENTED_EDGE('',*,*,#51026,.F.);
#69327=ORIENTED_EDGE('',*,*,#49129,.F.);
#69328=ORIENTED_EDGE('',*,*,#51025,.T.);
#69329=ORIENTED_EDGE('',*,*,#49132,.F.);
#69330=ORIENTED_EDGE('',*,*,#51027,.F.);
#69331=ORIENTED_EDGE('',*,*,#47752,.F.);
#69332=ORIENTED_EDGE('',*,*,#51026,.T.);
#69333=ORIENTED_EDGE('',*,*,#47779,.F.);
#69334=ORIENTED_EDGE('',*,*,#51028,.F.);
#69335=ORIENTED_EDGE('',*,*,#49130,.F.);
#69336=ORIENTED_EDGE('',*,*,#51027,.T.);
#69337=ORIENTED_EDGE('',*,*,#49131,.F.);
#69338=ORIENTED_EDGE('',*,*,#51028,.T.);
#69339=ORIENTED_EDGE('',*,*,#47757,.F.);
#69340=ORIENTED_EDGE('',*,*,#47753,.T.);
#69341=ORIENTED_EDGE('',*,*,#51029,.F.);
#69342=ORIENTED_EDGE('',*,*,#49171,.F.);
#69343=ORIENTED_EDGE('',*,*,#51030,.F.);
#69344=ORIENTED_EDGE('',*,*,#47709,.F.);
#69345=ORIENTED_EDGE('',*,*,#51030,.T.);
#69346=ORIENTED_EDGE('',*,*,#49170,.F.);
#69347=ORIENTED_EDGE('',*,*,#51031,.F.);
#69348=ORIENTED_EDGE('',*,*,#47718,.F.);
#69349=ORIENTED_EDGE('',*,*,#47708,.T.);
#69350=ORIENTED_EDGE('',*,*,#47712,.F.);
#69351=ORIENTED_EDGE('',*,*,#51032,.F.);
#69352=ORIENTED_EDGE('',*,*,#49172,.F.);
#69353=ORIENTED_EDGE('',*,*,#51029,.T.);
#69354=ORIENTED_EDGE('',*,*,#51031,.T.);
#69355=ORIENTED_EDGE('',*,*,#49169,.F.);
#69356=ORIENTED_EDGE('',*,*,#51033,.F.);
#69357=ORIENTED_EDGE('',*,*,#47703,.F.);
#69358=ORIENTED_EDGE('',*,*,#51032,.T.);
#69359=ORIENTED_EDGE('',*,*,#47716,.F.);
#69360=ORIENTED_EDGE('',*,*,#51034,.F.);
#69361=ORIENTED_EDGE('',*,*,#49161,.F.);
#69362=ORIENTED_EDGE('',*,*,#51033,.T.);
#69363=ORIENTED_EDGE('',*,*,#49168,.F.);
#69364=ORIENTED_EDGE('',*,*,#51035,.F.);
#69365=ORIENTED_EDGE('',*,*,#47720,.F.);
#69366=ORIENTED_EDGE('',*,*,#51034,.T.);
#69367=ORIENTED_EDGE('',*,*,#46063,.F.);
#69368=ORIENTED_EDGE('',*,*,#51036,.F.);
#69369=ORIENTED_EDGE('',*,*,#49162,.F.);
#69370=ORIENTED_EDGE('',*,*,#51035,.T.);
#69371=ORIENTED_EDGE('',*,*,#49167,.F.);
#69372=ORIENTED_EDGE('',*,*,#51037,.F.);
#69373=ORIENTED_EDGE('',*,*,#47695,.T.);
#69374=ORIENTED_EDGE('',*,*,#47699,.F.);
#69375=ORIENTED_EDGE('',*,*,#51036,.T.);
#69376=ORIENTED_EDGE('',*,*,#46062,.F.);
#69377=ORIENTED_EDGE('',*,*,#51038,.F.);
#69378=ORIENTED_EDGE('',*,*,#50241,.F.);
#69379=ORIENTED_EDGE('',*,*,#51037,.T.);
#69380=ORIENTED_EDGE('',*,*,#49166,.F.);
#69381=ORIENTED_EDGE('',*,*,#51039,.F.);
#69382=ORIENTED_EDGE('',*,*,#47696,.F.);
#69383=ORIENTED_EDGE('',*,*,#51038,.T.);
#69384=ORIENTED_EDGE('',*,*,#46061,.F.);
#69385=ORIENTED_EDGE('',*,*,#51040,.F.);
#69386=ORIENTED_EDGE('',*,*,#49146,.F.);
#69387=ORIENTED_EDGE('',*,*,#51039,.T.);
#69388=ORIENTED_EDGE('',*,*,#49165,.F.);
#69389=ORIENTED_EDGE('',*,*,#51041,.F.);
#69390=ORIENTED_EDGE('',*,*,#47714,.F.);
#69391=ORIENTED_EDGE('',*,*,#51040,.T.);
#69392=ORIENTED_EDGE('',*,*,#46060,.F.);
#69393=ORIENTED_EDGE('',*,*,#51042,.F.);
#69394=ORIENTED_EDGE('',*,*,#50243,.F.);
#69395=ORIENTED_EDGE('',*,*,#51041,.T.);
#69396=ORIENTED_EDGE('',*,*,#49164,.F.);
#69397=ORIENTED_EDGE('',*,*,#51043,.F.);
#69398=ORIENTED_EDGE('',*,*,#46309,.F.);
#69399=ORIENTED_EDGE('',*,*,#51042,.T.);
#69400=ORIENTED_EDGE('',*,*,#46059,.F.);
#69401=ORIENTED_EDGE('',*,*,#51044,.F.);
#69402=ORIENTED_EDGE('',*,*,#49152,.F.);
#69403=ORIENTED_EDGE('',*,*,#51043,.T.);
#69404=ORIENTED_EDGE('',*,*,#50242,.F.);
#69405=ORIENTED_EDGE('',*,*,#51045,.F.);
#69406=ORIENTED_EDGE('',*,*,#46310,.F.);
#69407=ORIENTED_EDGE('',*,*,#51044,.T.);
#69408=ORIENTED_EDGE('',*,*,#47745,.F.);
#69409=ORIENTED_EDGE('',*,*,#51046,.F.);
#69410=ORIENTED_EDGE('',*,*,#49153,.F.);
#69411=ORIENTED_EDGE('',*,*,#51045,.T.);
#69412=ORIENTED_EDGE('',*,*,#49148,.F.);
#69413=ORIENTED_EDGE('',*,*,#51047,.F.);
#69414=ORIENTED_EDGE('',*,*,#46311,.F.);
#69415=ORIENTED_EDGE('',*,*,#47740,.F.);
#69416=ORIENTED_EDGE('',*,*,#47736,.T.);
#69417=ORIENTED_EDGE('',*,*,#51048,.F.);
#69418=ORIENTED_EDGE('',*,*,#49154,.F.);
#69419=ORIENTED_EDGE('',*,*,#51046,.T.);
#69420=ORIENTED_EDGE('',*,*,#51047,.T.);
#69421=ORIENTED_EDGE('',*,*,#50244,.F.);
#69422=ORIENTED_EDGE('',*,*,#51049,.F.);
#69423=ORIENTED_EDGE('',*,*,#46312,.F.);
#69424=ORIENTED_EDGE('',*,*,#51048,.T.);
#69425=ORIENTED_EDGE('',*,*,#47735,.F.);
#69426=ORIENTED_EDGE('',*,*,#51050,.F.);
#69427=ORIENTED_EDGE('',*,*,#49155,.F.);
#69428=ORIENTED_EDGE('',*,*,#51049,.T.);
#69429=ORIENTED_EDGE('',*,*,#49150,.F.);
#69430=ORIENTED_EDGE('',*,*,#51051,.F.);
#69431=ORIENTED_EDGE('',*,*,#46313,.F.);
#69432=ORIENTED_EDGE('',*,*,#51050,.T.);
#69433=ORIENTED_EDGE('',*,*,#47747,.F.);
#69434=ORIENTED_EDGE('',*,*,#51052,.F.);
#69435=ORIENTED_EDGE('',*,*,#49156,.F.);
#69436=ORIENTED_EDGE('',*,*,#51051,.T.);
#69437=ORIENTED_EDGE('',*,*,#49149,.F.);
#69438=ORIENTED_EDGE('',*,*,#51053,.F.);
#69439=ORIENTED_EDGE('',*,*,#47743,.F.);
#69440=ORIENTED_EDGE('',*,*,#51052,.T.);
#69441=ORIENTED_EDGE('',*,*,#47731,.F.);
#69442=ORIENTED_EDGE('',*,*,#51054,.F.);
#69443=ORIENTED_EDGE('',*,*,#49157,.F.);
#69444=ORIENTED_EDGE('',*,*,#51053,.T.);
#69445=ORIENTED_EDGE('',*,*,#49160,.F.);
#69446=ORIENTED_EDGE('',*,*,#51055,.F.);
#69447=ORIENTED_EDGE('',*,*,#47722,.F.);
#69448=ORIENTED_EDGE('',*,*,#51054,.T.);
#69449=ORIENTED_EDGE('',*,*,#47749,.F.);
#69450=ORIENTED_EDGE('',*,*,#51056,.F.);
#69451=ORIENTED_EDGE('',*,*,#49158,.F.);
#69452=ORIENTED_EDGE('',*,*,#51055,.T.);
#69453=ORIENTED_EDGE('',*,*,#49159,.F.);
#69454=ORIENTED_EDGE('',*,*,#51056,.T.);
#69455=ORIENTED_EDGE('',*,*,#47727,.F.);
#69456=ORIENTED_EDGE('',*,*,#47723,.T.);
#69457=ORIENTED_EDGE('',*,*,#51057,.F.);
#69458=ORIENTED_EDGE('',*,*,#49199,.F.);
#69459=ORIENTED_EDGE('',*,*,#51058,.F.);
#69460=ORIENTED_EDGE('',*,*,#47679,.F.);
#69461=ORIENTED_EDGE('',*,*,#51058,.T.);
#69462=ORIENTED_EDGE('',*,*,#49198,.F.);
#69463=ORIENTED_EDGE('',*,*,#51059,.F.);
#69464=ORIENTED_EDGE('',*,*,#47688,.F.);
#69465=ORIENTED_EDGE('',*,*,#47678,.T.);
#69466=ORIENTED_EDGE('',*,*,#47682,.F.);
#69467=ORIENTED_EDGE('',*,*,#51060,.F.);
#69468=ORIENTED_EDGE('',*,*,#49200,.F.);
#69469=ORIENTED_EDGE('',*,*,#51057,.T.);
#69470=ORIENTED_EDGE('',*,*,#51059,.T.);
#69471=ORIENTED_EDGE('',*,*,#49197,.F.);
#69472=ORIENTED_EDGE('',*,*,#51061,.F.);
#69473=ORIENTED_EDGE('',*,*,#47673,.F.);
#69474=ORIENTED_EDGE('',*,*,#51060,.T.);
#69475=ORIENTED_EDGE('',*,*,#47686,.F.);
#69476=ORIENTED_EDGE('',*,*,#51062,.F.);
#69477=ORIENTED_EDGE('',*,*,#49189,.F.);
#69478=ORIENTED_EDGE('',*,*,#51061,.T.);
#69479=ORIENTED_EDGE('',*,*,#49196,.F.);
#69480=ORIENTED_EDGE('',*,*,#51063,.F.);
#69481=ORIENTED_EDGE('',*,*,#47690,.F.);
#69482=ORIENTED_EDGE('',*,*,#51062,.T.);
#69483=ORIENTED_EDGE('',*,*,#46069,.F.);
#69484=ORIENTED_EDGE('',*,*,#51064,.F.);
#69485=ORIENTED_EDGE('',*,*,#49190,.F.);
#69486=ORIENTED_EDGE('',*,*,#51063,.T.);
#69487=ORIENTED_EDGE('',*,*,#49195,.F.);
#69488=ORIENTED_EDGE('',*,*,#51065,.F.);
#69489=ORIENTED_EDGE('',*,*,#47665,.T.);
#69490=ORIENTED_EDGE('',*,*,#47669,.F.);
#69491=ORIENTED_EDGE('',*,*,#51064,.T.);
#69492=ORIENTED_EDGE('',*,*,#46068,.F.);
#69493=ORIENTED_EDGE('',*,*,#51066,.F.);
#69494=ORIENTED_EDGE('',*,*,#50245,.F.);
#69495=ORIENTED_EDGE('',*,*,#51065,.T.);
#69496=ORIENTED_EDGE('',*,*,#49194,.F.);
#69497=ORIENTED_EDGE('',*,*,#51067,.F.);
#69498=ORIENTED_EDGE('',*,*,#47666,.F.);
#69499=ORIENTED_EDGE('',*,*,#51066,.T.);
#69500=ORIENTED_EDGE('',*,*,#46067,.F.);
#69501=ORIENTED_EDGE('',*,*,#51068,.F.);
#69502=ORIENTED_EDGE('',*,*,#49174,.F.);
#69503=ORIENTED_EDGE('',*,*,#51067,.T.);
#69504=ORIENTED_EDGE('',*,*,#49193,.F.);
#69505=ORIENTED_EDGE('',*,*,#51069,.F.);
#69506=ORIENTED_EDGE('',*,*,#47684,.F.);
#69507=ORIENTED_EDGE('',*,*,#51068,.T.);
#69508=ORIENTED_EDGE('',*,*,#46066,.F.);
#69509=ORIENTED_EDGE('',*,*,#51070,.F.);
#69510=ORIENTED_EDGE('',*,*,#50247,.F.);
#69511=ORIENTED_EDGE('',*,*,#51069,.T.);
#69512=ORIENTED_EDGE('',*,*,#49192,.F.);
#69513=ORIENTED_EDGE('',*,*,#51071,.F.);
#69514=ORIENTED_EDGE('',*,*,#46303,.F.);
#69515=ORIENTED_EDGE('',*,*,#51070,.T.);
#69516=ORIENTED_EDGE('',*,*,#46065,.F.);
#69517=ORIENTED_EDGE('',*,*,#51072,.F.);
#69518=ORIENTED_EDGE('',*,*,#49180,.F.);
#69519=ORIENTED_EDGE('',*,*,#51071,.T.);
#69520=ORIENTED_EDGE('',*,*,#50246,.F.);
#69521=ORIENTED_EDGE('',*,*,#51073,.F.);
#69522=ORIENTED_EDGE('',*,*,#46304,.F.);
#69523=ORIENTED_EDGE('',*,*,#51072,.T.);
#69524=ORIENTED_EDGE('',*,*,#47715,.F.);
#69525=ORIENTED_EDGE('',*,*,#51074,.F.);
#69526=ORIENTED_EDGE('',*,*,#49181,.F.);
#69527=ORIENTED_EDGE('',*,*,#51073,.T.);
#69528=ORIENTED_EDGE('',*,*,#49176,.F.);
#69529=ORIENTED_EDGE('',*,*,#51075,.F.);
#69530=ORIENTED_EDGE('',*,*,#46305,.F.);
#69531=ORIENTED_EDGE('',*,*,#47710,.F.);
#69532=ORIENTED_EDGE('',*,*,#47706,.T.);
#69533=ORIENTED_EDGE('',*,*,#51076,.F.);
#69534=ORIENTED_EDGE('',*,*,#49182,.F.);
#69535=ORIENTED_EDGE('',*,*,#51074,.T.);
#69536=ORIENTED_EDGE('',*,*,#51075,.T.);
#69537=ORIENTED_EDGE('',*,*,#50248,.F.);
#69538=ORIENTED_EDGE('',*,*,#51077,.F.);
#69539=ORIENTED_EDGE('',*,*,#46306,.F.);
#69540=ORIENTED_EDGE('',*,*,#51076,.T.);
#69541=ORIENTED_EDGE('',*,*,#47705,.F.);
#69542=ORIENTED_EDGE('',*,*,#51078,.F.);
#69543=ORIENTED_EDGE('',*,*,#49183,.F.);
#69544=ORIENTED_EDGE('',*,*,#51077,.T.);
#69545=ORIENTED_EDGE('',*,*,#49178,.F.);
#69546=ORIENTED_EDGE('',*,*,#51079,.F.);
#69547=ORIENTED_EDGE('',*,*,#46307,.F.);
#69548=ORIENTED_EDGE('',*,*,#51078,.T.);
#69549=ORIENTED_EDGE('',*,*,#47717,.F.);
#69550=ORIENTED_EDGE('',*,*,#51080,.F.);
#69551=ORIENTED_EDGE('',*,*,#49184,.F.);
#69552=ORIENTED_EDGE('',*,*,#51079,.T.);
#69553=ORIENTED_EDGE('',*,*,#49177,.F.);
#69554=ORIENTED_EDGE('',*,*,#51081,.F.);
#69555=ORIENTED_EDGE('',*,*,#47713,.F.);
#69556=ORIENTED_EDGE('',*,*,#51080,.T.);
#69557=ORIENTED_EDGE('',*,*,#47701,.F.);
#69558=ORIENTED_EDGE('',*,*,#51082,.F.);
#69559=ORIENTED_EDGE('',*,*,#49185,.F.);
#69560=ORIENTED_EDGE('',*,*,#51081,.T.);
#69561=ORIENTED_EDGE('',*,*,#49188,.F.);
#69562=ORIENTED_EDGE('',*,*,#51083,.F.);
#69563=ORIENTED_EDGE('',*,*,#47692,.F.);
#69564=ORIENTED_EDGE('',*,*,#51082,.T.);
#69565=ORIENTED_EDGE('',*,*,#47719,.F.);
#69566=ORIENTED_EDGE('',*,*,#51084,.F.);
#69567=ORIENTED_EDGE('',*,*,#49186,.F.);
#69568=ORIENTED_EDGE('',*,*,#51083,.T.);
#69569=ORIENTED_EDGE('',*,*,#49187,.F.);
#69570=ORIENTED_EDGE('',*,*,#51084,.T.);
#69571=ORIENTED_EDGE('',*,*,#47697,.F.);
#69572=ORIENTED_EDGE('',*,*,#47693,.T.);
#69573=ORIENTED_EDGE('',*,*,#51085,.F.);
#69574=ORIENTED_EDGE('',*,*,#49227,.F.);
#69575=ORIENTED_EDGE('',*,*,#51086,.F.);
#69576=ORIENTED_EDGE('',*,*,#47649,.F.);
#69577=ORIENTED_EDGE('',*,*,#51086,.T.);
#69578=ORIENTED_EDGE('',*,*,#49226,.F.);
#69579=ORIENTED_EDGE('',*,*,#51087,.F.);
#69580=ORIENTED_EDGE('',*,*,#47658,.F.);
#69581=ORIENTED_EDGE('',*,*,#47648,.T.);
#69582=ORIENTED_EDGE('',*,*,#47652,.F.);
#69583=ORIENTED_EDGE('',*,*,#51088,.F.);
#69584=ORIENTED_EDGE('',*,*,#49228,.F.);
#69585=ORIENTED_EDGE('',*,*,#51085,.T.);
#69586=ORIENTED_EDGE('',*,*,#51087,.T.);
#69587=ORIENTED_EDGE('',*,*,#49225,.F.);
#69588=ORIENTED_EDGE('',*,*,#51089,.F.);
#69589=ORIENTED_EDGE('',*,*,#47643,.F.);
#69590=ORIENTED_EDGE('',*,*,#51088,.T.);
#69591=ORIENTED_EDGE('',*,*,#47656,.F.);
#69592=ORIENTED_EDGE('',*,*,#51090,.F.);
#69593=ORIENTED_EDGE('',*,*,#49217,.F.);
#69594=ORIENTED_EDGE('',*,*,#51089,.T.);
#69595=ORIENTED_EDGE('',*,*,#49224,.F.);
#69596=ORIENTED_EDGE('',*,*,#51091,.F.);
#69597=ORIENTED_EDGE('',*,*,#47660,.F.);
#69598=ORIENTED_EDGE('',*,*,#51090,.T.);
#69599=ORIENTED_EDGE('',*,*,#46075,.F.);
#69600=ORIENTED_EDGE('',*,*,#51092,.F.);
#69601=ORIENTED_EDGE('',*,*,#49218,.F.);
#69602=ORIENTED_EDGE('',*,*,#51091,.T.);
#69603=ORIENTED_EDGE('',*,*,#49223,.F.);
#69604=ORIENTED_EDGE('',*,*,#51093,.F.);
#69605=ORIENTED_EDGE('',*,*,#47635,.T.);
#69606=ORIENTED_EDGE('',*,*,#47639,.F.);
#69607=ORIENTED_EDGE('',*,*,#51092,.T.);
#69608=ORIENTED_EDGE('',*,*,#46074,.F.);
#69609=ORIENTED_EDGE('',*,*,#51094,.F.);
#69610=ORIENTED_EDGE('',*,*,#50249,.F.);
#69611=ORIENTED_EDGE('',*,*,#51093,.T.);
#69612=ORIENTED_EDGE('',*,*,#49222,.F.);
#69613=ORIENTED_EDGE('',*,*,#51095,.F.);
#69614=ORIENTED_EDGE('',*,*,#47636,.F.);
#69615=ORIENTED_EDGE('',*,*,#51094,.T.);
#69616=ORIENTED_EDGE('',*,*,#46073,.F.);
#69617=ORIENTED_EDGE('',*,*,#51096,.F.);
#69618=ORIENTED_EDGE('',*,*,#49202,.F.);
#69619=ORIENTED_EDGE('',*,*,#51095,.T.);
#69620=ORIENTED_EDGE('',*,*,#49221,.F.);
#69621=ORIENTED_EDGE('',*,*,#51097,.F.);
#69622=ORIENTED_EDGE('',*,*,#47654,.F.);
#69623=ORIENTED_EDGE('',*,*,#51096,.T.);
#69624=ORIENTED_EDGE('',*,*,#46072,.F.);
#69625=ORIENTED_EDGE('',*,*,#51098,.F.);
#69626=ORIENTED_EDGE('',*,*,#50251,.F.);
#69627=ORIENTED_EDGE('',*,*,#51097,.T.);
#69628=ORIENTED_EDGE('',*,*,#49220,.F.);
#69629=ORIENTED_EDGE('',*,*,#51099,.F.);
#69630=ORIENTED_EDGE('',*,*,#46297,.F.);
#69631=ORIENTED_EDGE('',*,*,#51098,.T.);
#69632=ORIENTED_EDGE('',*,*,#46071,.F.);
#69633=ORIENTED_EDGE('',*,*,#51100,.F.);
#69634=ORIENTED_EDGE('',*,*,#49208,.F.);
#69635=ORIENTED_EDGE('',*,*,#51099,.T.);
#69636=ORIENTED_EDGE('',*,*,#50250,.F.);
#69637=ORIENTED_EDGE('',*,*,#51101,.F.);
#69638=ORIENTED_EDGE('',*,*,#46298,.F.);
#69639=ORIENTED_EDGE('',*,*,#51100,.T.);
#69640=ORIENTED_EDGE('',*,*,#47685,.F.);
#69641=ORIENTED_EDGE('',*,*,#51102,.F.);
#69642=ORIENTED_EDGE('',*,*,#49209,.F.);
#69643=ORIENTED_EDGE('',*,*,#51101,.T.);
#69644=ORIENTED_EDGE('',*,*,#49204,.F.);
#69645=ORIENTED_EDGE('',*,*,#51103,.F.);
#69646=ORIENTED_EDGE('',*,*,#46299,.F.);
#69647=ORIENTED_EDGE('',*,*,#47680,.F.);
#69648=ORIENTED_EDGE('',*,*,#47676,.T.);
#69649=ORIENTED_EDGE('',*,*,#51104,.F.);
#69650=ORIENTED_EDGE('',*,*,#49210,.F.);
#69651=ORIENTED_EDGE('',*,*,#51102,.T.);
#69652=ORIENTED_EDGE('',*,*,#51103,.T.);
#69653=ORIENTED_EDGE('',*,*,#50252,.F.);
#69654=ORIENTED_EDGE('',*,*,#51105,.F.);
#69655=ORIENTED_EDGE('',*,*,#46300,.F.);
#69656=ORIENTED_EDGE('',*,*,#51104,.T.);
#69657=ORIENTED_EDGE('',*,*,#47675,.F.);
#69658=ORIENTED_EDGE('',*,*,#51106,.F.);
#69659=ORIENTED_EDGE('',*,*,#49211,.F.);
#69660=ORIENTED_EDGE('',*,*,#51105,.T.);
#69661=ORIENTED_EDGE('',*,*,#49206,.F.);
#69662=ORIENTED_EDGE('',*,*,#51107,.F.);
#69663=ORIENTED_EDGE('',*,*,#46301,.F.);
#69664=ORIENTED_EDGE('',*,*,#51106,.T.);
#69665=ORIENTED_EDGE('',*,*,#47687,.F.);
#69666=ORIENTED_EDGE('',*,*,#51108,.F.);
#69667=ORIENTED_EDGE('',*,*,#49212,.F.);
#69668=ORIENTED_EDGE('',*,*,#51107,.T.);
#69669=ORIENTED_EDGE('',*,*,#49205,.F.);
#69670=ORIENTED_EDGE('',*,*,#51109,.F.);
#69671=ORIENTED_EDGE('',*,*,#47683,.F.);
#69672=ORIENTED_EDGE('',*,*,#51108,.T.);
#69673=ORIENTED_EDGE('',*,*,#47671,.F.);
#69674=ORIENTED_EDGE('',*,*,#51110,.F.);
#69675=ORIENTED_EDGE('',*,*,#49213,.F.);
#69676=ORIENTED_EDGE('',*,*,#51109,.T.);
#69677=ORIENTED_EDGE('',*,*,#49216,.F.);
#69678=ORIENTED_EDGE('',*,*,#51111,.F.);
#69679=ORIENTED_EDGE('',*,*,#47662,.F.);
#69680=ORIENTED_EDGE('',*,*,#51110,.T.);
#69681=ORIENTED_EDGE('',*,*,#47689,.F.);
#69682=ORIENTED_EDGE('',*,*,#51112,.F.);
#69683=ORIENTED_EDGE('',*,*,#49214,.F.);
#69684=ORIENTED_EDGE('',*,*,#51111,.T.);
#69685=ORIENTED_EDGE('',*,*,#49215,.F.);
#69686=ORIENTED_EDGE('',*,*,#51112,.T.);
#69687=ORIENTED_EDGE('',*,*,#47667,.F.);
#69688=ORIENTED_EDGE('',*,*,#47663,.T.);
#69689=ORIENTED_EDGE('',*,*,#51113,.F.);
#69690=ORIENTED_EDGE('',*,*,#49255,.F.);
#69691=ORIENTED_EDGE('',*,*,#51114,.F.);
#69692=ORIENTED_EDGE('',*,*,#47619,.F.);
#69693=ORIENTED_EDGE('',*,*,#51114,.T.);
#69694=ORIENTED_EDGE('',*,*,#49254,.F.);
#69695=ORIENTED_EDGE('',*,*,#51115,.F.);
#69696=ORIENTED_EDGE('',*,*,#47628,.F.);
#69697=ORIENTED_EDGE('',*,*,#47618,.T.);
#69698=ORIENTED_EDGE('',*,*,#47622,.F.);
#69699=ORIENTED_EDGE('',*,*,#51116,.F.);
#69700=ORIENTED_EDGE('',*,*,#49256,.F.);
#69701=ORIENTED_EDGE('',*,*,#51113,.T.);
#69702=ORIENTED_EDGE('',*,*,#51115,.T.);
#69703=ORIENTED_EDGE('',*,*,#49253,.F.);
#69704=ORIENTED_EDGE('',*,*,#51117,.F.);
#69705=ORIENTED_EDGE('',*,*,#47613,.F.);
#69706=ORIENTED_EDGE('',*,*,#51116,.T.);
#69707=ORIENTED_EDGE('',*,*,#47626,.F.);
#69708=ORIENTED_EDGE('',*,*,#51118,.F.);
#69709=ORIENTED_EDGE('',*,*,#49245,.F.);
#69710=ORIENTED_EDGE('',*,*,#51117,.T.);
#69711=ORIENTED_EDGE('',*,*,#49252,.F.);
#69712=ORIENTED_EDGE('',*,*,#51119,.F.);
#69713=ORIENTED_EDGE('',*,*,#47630,.F.);
#69714=ORIENTED_EDGE('',*,*,#51118,.T.);
#69715=ORIENTED_EDGE('',*,*,#46081,.F.);
#69716=ORIENTED_EDGE('',*,*,#51120,.F.);
#69717=ORIENTED_EDGE('',*,*,#49246,.F.);
#69718=ORIENTED_EDGE('',*,*,#51119,.T.);
#69719=ORIENTED_EDGE('',*,*,#49251,.F.);
#69720=ORIENTED_EDGE('',*,*,#51121,.F.);
#69721=ORIENTED_EDGE('',*,*,#47605,.T.);
#69722=ORIENTED_EDGE('',*,*,#47609,.F.);
#69723=ORIENTED_EDGE('',*,*,#51120,.T.);
#69724=ORIENTED_EDGE('',*,*,#46080,.F.);
#69725=ORIENTED_EDGE('',*,*,#51122,.F.);
#69726=ORIENTED_EDGE('',*,*,#50253,.F.);
#69727=ORIENTED_EDGE('',*,*,#51121,.T.);
#69728=ORIENTED_EDGE('',*,*,#49250,.F.);
#69729=ORIENTED_EDGE('',*,*,#51123,.F.);
#69730=ORIENTED_EDGE('',*,*,#47606,.F.);
#69731=ORIENTED_EDGE('',*,*,#51122,.T.);
#69732=ORIENTED_EDGE('',*,*,#46079,.F.);
#69733=ORIENTED_EDGE('',*,*,#51124,.F.);
#69734=ORIENTED_EDGE('',*,*,#49230,.F.);
#69735=ORIENTED_EDGE('',*,*,#51123,.T.);
#69736=ORIENTED_EDGE('',*,*,#49249,.F.);
#69737=ORIENTED_EDGE('',*,*,#51125,.F.);
#69738=ORIENTED_EDGE('',*,*,#47624,.F.);
#69739=ORIENTED_EDGE('',*,*,#51124,.T.);
#69740=ORIENTED_EDGE('',*,*,#46078,.F.);
#69741=ORIENTED_EDGE('',*,*,#51126,.F.);
#69742=ORIENTED_EDGE('',*,*,#50255,.F.);
#69743=ORIENTED_EDGE('',*,*,#51125,.T.);
#69744=ORIENTED_EDGE('',*,*,#49248,.F.);
#69745=ORIENTED_EDGE('',*,*,#51127,.F.);
#69746=ORIENTED_EDGE('',*,*,#46291,.F.);
#69747=ORIENTED_EDGE('',*,*,#51126,.T.);
#69748=ORIENTED_EDGE('',*,*,#46077,.F.);
#69749=ORIENTED_EDGE('',*,*,#51128,.F.);
#69750=ORIENTED_EDGE('',*,*,#49236,.F.);
#69751=ORIENTED_EDGE('',*,*,#51127,.T.);
#69752=ORIENTED_EDGE('',*,*,#50254,.F.);
#69753=ORIENTED_EDGE('',*,*,#51129,.F.);
#69754=ORIENTED_EDGE('',*,*,#46292,.F.);
#69755=ORIENTED_EDGE('',*,*,#51128,.T.);
#69756=ORIENTED_EDGE('',*,*,#47655,.F.);
#69757=ORIENTED_EDGE('',*,*,#51130,.F.);
#69758=ORIENTED_EDGE('',*,*,#49237,.F.);
#69759=ORIENTED_EDGE('',*,*,#51129,.T.);
#69760=ORIENTED_EDGE('',*,*,#49232,.F.);
#69761=ORIENTED_EDGE('',*,*,#51131,.F.);
#69762=ORIENTED_EDGE('',*,*,#46293,.F.);
#69763=ORIENTED_EDGE('',*,*,#47650,.F.);
#69764=ORIENTED_EDGE('',*,*,#47646,.T.);
#69765=ORIENTED_EDGE('',*,*,#51132,.F.);
#69766=ORIENTED_EDGE('',*,*,#49238,.F.);
#69767=ORIENTED_EDGE('',*,*,#51130,.T.);
#69768=ORIENTED_EDGE('',*,*,#51131,.T.);
#69769=ORIENTED_EDGE('',*,*,#50256,.F.);
#69770=ORIENTED_EDGE('',*,*,#51133,.F.);
#69771=ORIENTED_EDGE('',*,*,#46294,.F.);
#69772=ORIENTED_EDGE('',*,*,#51132,.T.);
#69773=ORIENTED_EDGE('',*,*,#47645,.F.);
#69774=ORIENTED_EDGE('',*,*,#51134,.F.);
#69775=ORIENTED_EDGE('',*,*,#49239,.F.);
#69776=ORIENTED_EDGE('',*,*,#51133,.T.);
#69777=ORIENTED_EDGE('',*,*,#49234,.F.);
#69778=ORIENTED_EDGE('',*,*,#51135,.F.);
#69779=ORIENTED_EDGE('',*,*,#46295,.F.);
#69780=ORIENTED_EDGE('',*,*,#51134,.T.);
#69781=ORIENTED_EDGE('',*,*,#47657,.F.);
#69782=ORIENTED_EDGE('',*,*,#51136,.F.);
#69783=ORIENTED_EDGE('',*,*,#49240,.F.);
#69784=ORIENTED_EDGE('',*,*,#51135,.T.);
#69785=ORIENTED_EDGE('',*,*,#49233,.F.);
#69786=ORIENTED_EDGE('',*,*,#51137,.F.);
#69787=ORIENTED_EDGE('',*,*,#47653,.F.);
#69788=ORIENTED_EDGE('',*,*,#51136,.T.);
#69789=ORIENTED_EDGE('',*,*,#47641,.F.);
#69790=ORIENTED_EDGE('',*,*,#51138,.F.);
#69791=ORIENTED_EDGE('',*,*,#49241,.F.);
#69792=ORIENTED_EDGE('',*,*,#51137,.T.);
#69793=ORIENTED_EDGE('',*,*,#49244,.F.);
#69794=ORIENTED_EDGE('',*,*,#51139,.F.);
#69795=ORIENTED_EDGE('',*,*,#47632,.F.);
#69796=ORIENTED_EDGE('',*,*,#51138,.T.);
#69797=ORIENTED_EDGE('',*,*,#47659,.F.);
#69798=ORIENTED_EDGE('',*,*,#51140,.F.);
#69799=ORIENTED_EDGE('',*,*,#49242,.F.);
#69800=ORIENTED_EDGE('',*,*,#51139,.T.);
#69801=ORIENTED_EDGE('',*,*,#49243,.F.);
#69802=ORIENTED_EDGE('',*,*,#51140,.T.);
#69803=ORIENTED_EDGE('',*,*,#47637,.F.);
#69804=ORIENTED_EDGE('',*,*,#47633,.T.);
#69805=ORIENTED_EDGE('',*,*,#51141,.F.);
#69806=ORIENTED_EDGE('',*,*,#49283,.F.);
#69807=ORIENTED_EDGE('',*,*,#51142,.F.);
#69808=ORIENTED_EDGE('',*,*,#47589,.F.);
#69809=ORIENTED_EDGE('',*,*,#51142,.T.);
#69810=ORIENTED_EDGE('',*,*,#49282,.F.);
#69811=ORIENTED_EDGE('',*,*,#51143,.F.);
#69812=ORIENTED_EDGE('',*,*,#47598,.F.);
#69813=ORIENTED_EDGE('',*,*,#47588,.T.);
#69814=ORIENTED_EDGE('',*,*,#47592,.F.);
#69815=ORIENTED_EDGE('',*,*,#51144,.F.);
#69816=ORIENTED_EDGE('',*,*,#49284,.F.);
#69817=ORIENTED_EDGE('',*,*,#51141,.T.);
#69818=ORIENTED_EDGE('',*,*,#51143,.T.);
#69819=ORIENTED_EDGE('',*,*,#49281,.F.);
#69820=ORIENTED_EDGE('',*,*,#51145,.F.);
#69821=ORIENTED_EDGE('',*,*,#47583,.F.);
#69822=ORIENTED_EDGE('',*,*,#51144,.T.);
#69823=ORIENTED_EDGE('',*,*,#47596,.F.);
#69824=ORIENTED_EDGE('',*,*,#51146,.F.);
#69825=ORIENTED_EDGE('',*,*,#49273,.F.);
#69826=ORIENTED_EDGE('',*,*,#51145,.T.);
#69827=ORIENTED_EDGE('',*,*,#49280,.F.);
#69828=ORIENTED_EDGE('',*,*,#51147,.F.);
#69829=ORIENTED_EDGE('',*,*,#47600,.F.);
#69830=ORIENTED_EDGE('',*,*,#51146,.T.);
#69831=ORIENTED_EDGE('',*,*,#46087,.F.);
#69832=ORIENTED_EDGE('',*,*,#51148,.F.);
#69833=ORIENTED_EDGE('',*,*,#49274,.F.);
#69834=ORIENTED_EDGE('',*,*,#51147,.T.);
#69835=ORIENTED_EDGE('',*,*,#49279,.F.);
#69836=ORIENTED_EDGE('',*,*,#51149,.F.);
#69837=ORIENTED_EDGE('',*,*,#47575,.T.);
#69838=ORIENTED_EDGE('',*,*,#47579,.F.);
#69839=ORIENTED_EDGE('',*,*,#51148,.T.);
#69840=ORIENTED_EDGE('',*,*,#46086,.F.);
#69841=ORIENTED_EDGE('',*,*,#51150,.F.);
#69842=ORIENTED_EDGE('',*,*,#50257,.F.);
#69843=ORIENTED_EDGE('',*,*,#51149,.T.);
#69844=ORIENTED_EDGE('',*,*,#49278,.F.);
#69845=ORIENTED_EDGE('',*,*,#51151,.F.);
#69846=ORIENTED_EDGE('',*,*,#47576,.F.);
#69847=ORIENTED_EDGE('',*,*,#51150,.T.);
#69848=ORIENTED_EDGE('',*,*,#46085,.F.);
#69849=ORIENTED_EDGE('',*,*,#51152,.F.);
#69850=ORIENTED_EDGE('',*,*,#49258,.F.);
#69851=ORIENTED_EDGE('',*,*,#51151,.T.);
#69852=ORIENTED_EDGE('',*,*,#49277,.F.);
#69853=ORIENTED_EDGE('',*,*,#51153,.F.);
#69854=ORIENTED_EDGE('',*,*,#47594,.F.);
#69855=ORIENTED_EDGE('',*,*,#51152,.T.);
#69856=ORIENTED_EDGE('',*,*,#46084,.F.);
#69857=ORIENTED_EDGE('',*,*,#51154,.F.);
#69858=ORIENTED_EDGE('',*,*,#50259,.F.);
#69859=ORIENTED_EDGE('',*,*,#51153,.T.);
#69860=ORIENTED_EDGE('',*,*,#49276,.F.);
#69861=ORIENTED_EDGE('',*,*,#51155,.F.);
#69862=ORIENTED_EDGE('',*,*,#46285,.F.);
#69863=ORIENTED_EDGE('',*,*,#51154,.T.);
#69864=ORIENTED_EDGE('',*,*,#46083,.F.);
#69865=ORIENTED_EDGE('',*,*,#51156,.F.);
#69866=ORIENTED_EDGE('',*,*,#49264,.F.);
#69867=ORIENTED_EDGE('',*,*,#51155,.T.);
#69868=ORIENTED_EDGE('',*,*,#50258,.F.);
#69869=ORIENTED_EDGE('',*,*,#51157,.F.);
#69870=ORIENTED_EDGE('',*,*,#46286,.F.);
#69871=ORIENTED_EDGE('',*,*,#51156,.T.);
#69872=ORIENTED_EDGE('',*,*,#47625,.F.);
#69873=ORIENTED_EDGE('',*,*,#51158,.F.);
#69874=ORIENTED_EDGE('',*,*,#49265,.F.);
#69875=ORIENTED_EDGE('',*,*,#51157,.T.);
#69876=ORIENTED_EDGE('',*,*,#49260,.F.);
#69877=ORIENTED_EDGE('',*,*,#51159,.F.);
#69878=ORIENTED_EDGE('',*,*,#46287,.F.);
#69879=ORIENTED_EDGE('',*,*,#47620,.F.);
#69880=ORIENTED_EDGE('',*,*,#47616,.T.);
#69881=ORIENTED_EDGE('',*,*,#51160,.F.);
#69882=ORIENTED_EDGE('',*,*,#49266,.F.);
#69883=ORIENTED_EDGE('',*,*,#51158,.T.);
#69884=ORIENTED_EDGE('',*,*,#51159,.T.);
#69885=ORIENTED_EDGE('',*,*,#50260,.F.);
#69886=ORIENTED_EDGE('',*,*,#51161,.F.);
#69887=ORIENTED_EDGE('',*,*,#46288,.F.);
#69888=ORIENTED_EDGE('',*,*,#51160,.T.);
#69889=ORIENTED_EDGE('',*,*,#47615,.F.);
#69890=ORIENTED_EDGE('',*,*,#51162,.F.);
#69891=ORIENTED_EDGE('',*,*,#49267,.F.);
#69892=ORIENTED_EDGE('',*,*,#51161,.T.);
#69893=ORIENTED_EDGE('',*,*,#49262,.F.);
#69894=ORIENTED_EDGE('',*,*,#51163,.F.);
#69895=ORIENTED_EDGE('',*,*,#46289,.F.);
#69896=ORIENTED_EDGE('',*,*,#51162,.T.);
#69897=ORIENTED_EDGE('',*,*,#47627,.F.);
#69898=ORIENTED_EDGE('',*,*,#51164,.F.);
#69899=ORIENTED_EDGE('',*,*,#49268,.F.);
#69900=ORIENTED_EDGE('',*,*,#51163,.T.);
#69901=ORIENTED_EDGE('',*,*,#49261,.F.);
#69902=ORIENTED_EDGE('',*,*,#51165,.F.);
#69903=ORIENTED_EDGE('',*,*,#47623,.F.);
#69904=ORIENTED_EDGE('',*,*,#51164,.T.);
#69905=ORIENTED_EDGE('',*,*,#47611,.F.);
#69906=ORIENTED_EDGE('',*,*,#51166,.F.);
#69907=ORIENTED_EDGE('',*,*,#49269,.F.);
#69908=ORIENTED_EDGE('',*,*,#51165,.T.);
#69909=ORIENTED_EDGE('',*,*,#49272,.F.);
#69910=ORIENTED_EDGE('',*,*,#51167,.F.);
#69911=ORIENTED_EDGE('',*,*,#47602,.F.);
#69912=ORIENTED_EDGE('',*,*,#51166,.T.);
#69913=ORIENTED_EDGE('',*,*,#47629,.F.);
#69914=ORIENTED_EDGE('',*,*,#51168,.F.);
#69915=ORIENTED_EDGE('',*,*,#49270,.F.);
#69916=ORIENTED_EDGE('',*,*,#51167,.T.);
#69917=ORIENTED_EDGE('',*,*,#49271,.F.);
#69918=ORIENTED_EDGE('',*,*,#51168,.T.);
#69919=ORIENTED_EDGE('',*,*,#47607,.F.);
#69920=ORIENTED_EDGE('',*,*,#47603,.T.);
#69921=ORIENTED_EDGE('',*,*,#51169,.F.);
#69922=ORIENTED_EDGE('',*,*,#49311,.F.);
#69923=ORIENTED_EDGE('',*,*,#51170,.F.);
#69924=ORIENTED_EDGE('',*,*,#47559,.F.);
#69925=ORIENTED_EDGE('',*,*,#51170,.T.);
#69926=ORIENTED_EDGE('',*,*,#49310,.F.);
#69927=ORIENTED_EDGE('',*,*,#51171,.F.);
#69928=ORIENTED_EDGE('',*,*,#47568,.F.);
#69929=ORIENTED_EDGE('',*,*,#47558,.T.);
#69930=ORIENTED_EDGE('',*,*,#47562,.F.);
#69931=ORIENTED_EDGE('',*,*,#51172,.F.);
#69932=ORIENTED_EDGE('',*,*,#49312,.F.);
#69933=ORIENTED_EDGE('',*,*,#51169,.T.);
#69934=ORIENTED_EDGE('',*,*,#51171,.T.);
#69935=ORIENTED_EDGE('',*,*,#49309,.F.);
#69936=ORIENTED_EDGE('',*,*,#51173,.F.);
#69937=ORIENTED_EDGE('',*,*,#47553,.F.);
#69938=ORIENTED_EDGE('',*,*,#51172,.T.);
#69939=ORIENTED_EDGE('',*,*,#47566,.F.);
#69940=ORIENTED_EDGE('',*,*,#51174,.F.);
#69941=ORIENTED_EDGE('',*,*,#49301,.F.);
#69942=ORIENTED_EDGE('',*,*,#51173,.T.);
#69943=ORIENTED_EDGE('',*,*,#49308,.F.);
#69944=ORIENTED_EDGE('',*,*,#51175,.F.);
#69945=ORIENTED_EDGE('',*,*,#47570,.F.);
#69946=ORIENTED_EDGE('',*,*,#51174,.T.);
#69947=ORIENTED_EDGE('',*,*,#46093,.F.);
#69948=ORIENTED_EDGE('',*,*,#51176,.F.);
#69949=ORIENTED_EDGE('',*,*,#49302,.F.);
#69950=ORIENTED_EDGE('',*,*,#51175,.T.);
#69951=ORIENTED_EDGE('',*,*,#49307,.F.);
#69952=ORIENTED_EDGE('',*,*,#51177,.F.);
#69953=ORIENTED_EDGE('',*,*,#47545,.T.);
#69954=ORIENTED_EDGE('',*,*,#47549,.F.);
#69955=ORIENTED_EDGE('',*,*,#51176,.T.);
#69956=ORIENTED_EDGE('',*,*,#46092,.F.);
#69957=ORIENTED_EDGE('',*,*,#51178,.F.);
#69958=ORIENTED_EDGE('',*,*,#50261,.F.);
#69959=ORIENTED_EDGE('',*,*,#51177,.T.);
#69960=ORIENTED_EDGE('',*,*,#49306,.F.);
#69961=ORIENTED_EDGE('',*,*,#51179,.F.);
#69962=ORIENTED_EDGE('',*,*,#47546,.F.);
#69963=ORIENTED_EDGE('',*,*,#51178,.T.);
#69964=ORIENTED_EDGE('',*,*,#46091,.F.);
#69965=ORIENTED_EDGE('',*,*,#51180,.F.);
#69966=ORIENTED_EDGE('',*,*,#49286,.F.);
#69967=ORIENTED_EDGE('',*,*,#51179,.T.);
#69968=ORIENTED_EDGE('',*,*,#49305,.F.);
#69969=ORIENTED_EDGE('',*,*,#51181,.F.);
#69970=ORIENTED_EDGE('',*,*,#47564,.F.);
#69971=ORIENTED_EDGE('',*,*,#51180,.T.);
#69972=ORIENTED_EDGE('',*,*,#46090,.F.);
#69973=ORIENTED_EDGE('',*,*,#51182,.F.);
#69974=ORIENTED_EDGE('',*,*,#50263,.F.);
#69975=ORIENTED_EDGE('',*,*,#51181,.T.);
#69976=ORIENTED_EDGE('',*,*,#49304,.F.);
#69977=ORIENTED_EDGE('',*,*,#51183,.F.);
#69978=ORIENTED_EDGE('',*,*,#46279,.F.);
#69979=ORIENTED_EDGE('',*,*,#51182,.T.);
#69980=ORIENTED_EDGE('',*,*,#46089,.F.);
#69981=ORIENTED_EDGE('',*,*,#51184,.F.);
#69982=ORIENTED_EDGE('',*,*,#49292,.F.);
#69983=ORIENTED_EDGE('',*,*,#51183,.T.);
#69984=ORIENTED_EDGE('',*,*,#50262,.F.);
#69985=ORIENTED_EDGE('',*,*,#51185,.F.);
#69986=ORIENTED_EDGE('',*,*,#46280,.F.);
#69987=ORIENTED_EDGE('',*,*,#51184,.T.);
#69988=ORIENTED_EDGE('',*,*,#47595,.F.);
#69989=ORIENTED_EDGE('',*,*,#51186,.F.);
#69990=ORIENTED_EDGE('',*,*,#49293,.F.);
#69991=ORIENTED_EDGE('',*,*,#51185,.T.);
#69992=ORIENTED_EDGE('',*,*,#49288,.F.);
#69993=ORIENTED_EDGE('',*,*,#51187,.F.);
#69994=ORIENTED_EDGE('',*,*,#46281,.F.);
#69995=ORIENTED_EDGE('',*,*,#47590,.F.);
#69996=ORIENTED_EDGE('',*,*,#47586,.T.);
#69997=ORIENTED_EDGE('',*,*,#51188,.F.);
#69998=ORIENTED_EDGE('',*,*,#49294,.F.);
#69999=ORIENTED_EDGE('',*,*,#51186,.T.);
#70000=ORIENTED_EDGE('',*,*,#51187,.T.);
#70001=ORIENTED_EDGE('',*,*,#50264,.F.);
#70002=ORIENTED_EDGE('',*,*,#51189,.F.);
#70003=ORIENTED_EDGE('',*,*,#46282,.F.);
#70004=ORIENTED_EDGE('',*,*,#51188,.T.);
#70005=ORIENTED_EDGE('',*,*,#47585,.F.);
#70006=ORIENTED_EDGE('',*,*,#51190,.F.);
#70007=ORIENTED_EDGE('',*,*,#49295,.F.);
#70008=ORIENTED_EDGE('',*,*,#51189,.T.);
#70009=ORIENTED_EDGE('',*,*,#49290,.F.);
#70010=ORIENTED_EDGE('',*,*,#51191,.F.);
#70011=ORIENTED_EDGE('',*,*,#46283,.F.);
#70012=ORIENTED_EDGE('',*,*,#51190,.T.);
#70013=ORIENTED_EDGE('',*,*,#47597,.F.);
#70014=ORIENTED_EDGE('',*,*,#51192,.F.);
#70015=ORIENTED_EDGE('',*,*,#49296,.F.);
#70016=ORIENTED_EDGE('',*,*,#51191,.T.);
#70017=ORIENTED_EDGE('',*,*,#49289,.F.);
#70018=ORIENTED_EDGE('',*,*,#51193,.F.);
#70019=ORIENTED_EDGE('',*,*,#47593,.F.);
#70020=ORIENTED_EDGE('',*,*,#51192,.T.);
#70021=ORIENTED_EDGE('',*,*,#47581,.F.);
#70022=ORIENTED_EDGE('',*,*,#51194,.F.);
#70023=ORIENTED_EDGE('',*,*,#49297,.F.);
#70024=ORIENTED_EDGE('',*,*,#51193,.T.);
#70025=ORIENTED_EDGE('',*,*,#49300,.F.);
#70026=ORIENTED_EDGE('',*,*,#51195,.F.);
#70027=ORIENTED_EDGE('',*,*,#47572,.F.);
#70028=ORIENTED_EDGE('',*,*,#51194,.T.);
#70029=ORIENTED_EDGE('',*,*,#47599,.F.);
#70030=ORIENTED_EDGE('',*,*,#51196,.F.);
#70031=ORIENTED_EDGE('',*,*,#49298,.F.);
#70032=ORIENTED_EDGE('',*,*,#51195,.T.);
#70033=ORIENTED_EDGE('',*,*,#49299,.F.);
#70034=ORIENTED_EDGE('',*,*,#51196,.T.);
#70035=ORIENTED_EDGE('',*,*,#47577,.F.);
#70036=ORIENTED_EDGE('',*,*,#47573,.T.);
#70037=ORIENTED_EDGE('',*,*,#51197,.F.);
#70038=ORIENTED_EDGE('',*,*,#49337,.F.);
#70039=ORIENTED_EDGE('',*,*,#51198,.F.);
#70040=ORIENTED_EDGE('',*,*,#47529,.F.);
#70041=ORIENTED_EDGE('',*,*,#51198,.T.);
#70042=ORIENTED_EDGE('',*,*,#49336,.F.);
#70043=ORIENTED_EDGE('',*,*,#51199,.F.);
#70044=ORIENTED_EDGE('',*,*,#47538,.F.);
#70045=ORIENTED_EDGE('',*,*,#47528,.T.);
#70046=ORIENTED_EDGE('',*,*,#47532,.F.);
#70047=ORIENTED_EDGE('',*,*,#51200,.F.);
#70048=ORIENTED_EDGE('',*,*,#49338,.F.);
#70049=ORIENTED_EDGE('',*,*,#51197,.T.);
#70050=ORIENTED_EDGE('',*,*,#51199,.T.);
#70051=ORIENTED_EDGE('',*,*,#49335,.F.);
#70052=ORIENTED_EDGE('',*,*,#51201,.F.);
#70053=ORIENTED_EDGE('',*,*,#47523,.F.);
#70054=ORIENTED_EDGE('',*,*,#51200,.T.);
#70055=ORIENTED_EDGE('',*,*,#47536,.F.);
#70056=ORIENTED_EDGE('',*,*,#51202,.F.);
#70057=ORIENTED_EDGE('',*,*,#49327,.F.);
#70058=ORIENTED_EDGE('',*,*,#51201,.T.);
#70059=ORIENTED_EDGE('',*,*,#49334,.F.);
#70060=ORIENTED_EDGE('',*,*,#51203,.F.);
#70061=ORIENTED_EDGE('',*,*,#47540,.F.);
#70062=ORIENTED_EDGE('',*,*,#51202,.T.);
#70063=ORIENTED_EDGE('',*,*,#46099,.F.);
#70064=ORIENTED_EDGE('',*,*,#51204,.F.);
#70065=ORIENTED_EDGE('',*,*,#49328,.F.);
#70066=ORIENTED_EDGE('',*,*,#51203,.T.);
#70067=ORIENTED_EDGE('',*,*,#49333,.F.);
#70068=ORIENTED_EDGE('',*,*,#51205,.F.);
#70069=ORIENTED_EDGE('',*,*,#47515,.T.);
#70070=ORIENTED_EDGE('',*,*,#47519,.F.);
#70071=ORIENTED_EDGE('',*,*,#51204,.T.);
#70072=ORIENTED_EDGE('',*,*,#46098,.F.);
#70073=ORIENTED_EDGE('',*,*,#45897,.F.);
#70074=ORIENTED_EDGE('',*,*,#50265,.F.);
#70075=ORIENTED_EDGE('',*,*,#51205,.T.);
#70076=ORIENTED_EDGE('',*,*,#49332,.F.);
#70077=ORIENTED_EDGE('',*,*,#51206,.F.);
#70078=ORIENTED_EDGE('',*,*,#47516,.F.);
#70079=ORIENTED_EDGE('',*,*,#51206,.T.);
#70080=ORIENTED_EDGE('',*,*,#49331,.F.);
#70081=ORIENTED_EDGE('',*,*,#51207,.F.);
#70082=ORIENTED_EDGE('',*,*,#47534,.F.);
#70083=ORIENTED_EDGE('',*,*,#45895,.T.);
#70084=ORIENTED_EDGE('',*,*,#46096,.F.);
#70085=ORIENTED_EDGE('',*,*,#51208,.F.);
#70086=ORIENTED_EDGE('',*,*,#50267,.F.);
#70087=ORIENTED_EDGE('',*,*,#51207,.T.);
#70088=ORIENTED_EDGE('',*,*,#49330,.F.);
#70089=ORIENTED_EDGE('',*,*,#51209,.F.);
#70090=ORIENTED_EDGE('',*,*,#46634,.F.);
#70091=ORIENTED_EDGE('',*,*,#51208,.T.);
#70092=ORIENTED_EDGE('',*,*,#46095,.F.);
#70093=ORIENTED_EDGE('',*,*,#51210,.F.);
#70094=ORIENTED_EDGE('',*,*,#49318,.F.);
#70095=ORIENTED_EDGE('',*,*,#51209,.T.);
#70096=ORIENTED_EDGE('',*,*,#50266,.F.);
#70097=ORIENTED_EDGE('',*,*,#45893,.F.);
#70098=ORIENTED_EDGE('',*,*,#46635,.F.);
#70099=ORIENTED_EDGE('',*,*,#51210,.T.);
#70100=ORIENTED_EDGE('',*,*,#47565,.F.);
#70101=ORIENTED_EDGE('',*,*,#51211,.F.);
#70102=ORIENTED_EDGE('',*,*,#49319,.F.);
#70103=ORIENTED_EDGE('',*,*,#47560,.F.);
#70104=ORIENTED_EDGE('',*,*,#47556,.T.);
#70105=ORIENTED_EDGE('',*,*,#51212,.F.);
#70106=ORIENTED_EDGE('',*,*,#49320,.F.);
#70107=ORIENTED_EDGE('',*,*,#51211,.T.);
#70108=ORIENTED_EDGE('',*,*,#45891,.T.);
#70109=ORIENTED_EDGE('',*,*,#50268,.F.);
#70110=ORIENTED_EDGE('',*,*,#51213,.F.);
#70111=ORIENTED_EDGE('',*,*,#46276,.F.);
#70112=ORIENTED_EDGE('',*,*,#51212,.T.);
#70113=ORIENTED_EDGE('',*,*,#47555,.F.);
#70114=ORIENTED_EDGE('',*,*,#51214,.F.);
#70115=ORIENTED_EDGE('',*,*,#49321,.F.);
#70116=ORIENTED_EDGE('',*,*,#51213,.T.);
#70117=ORIENTED_EDGE('',*,*,#49316,.F.);
#70118=ORIENTED_EDGE('',*,*,#51215,.F.);
#70119=ORIENTED_EDGE('',*,*,#46277,.F.);
#70120=ORIENTED_EDGE('',*,*,#51214,.T.);
#70121=ORIENTED_EDGE('',*,*,#47567,.F.);
#70122=ORIENTED_EDGE('',*,*,#51216,.F.);
#70123=ORIENTED_EDGE('',*,*,#49322,.F.);
#70124=ORIENTED_EDGE('',*,*,#51215,.T.);
#70125=ORIENTED_EDGE('',*,*,#49315,.F.);
#70126=ORIENTED_EDGE('',*,*,#51217,.F.);
#70127=ORIENTED_EDGE('',*,*,#47563,.F.);
#70128=ORIENTED_EDGE('',*,*,#51216,.T.);
#70129=ORIENTED_EDGE('',*,*,#47551,.F.);
#70130=ORIENTED_EDGE('',*,*,#51218,.F.);
#70131=ORIENTED_EDGE('',*,*,#49323,.F.);
#70132=ORIENTED_EDGE('',*,*,#51217,.T.);
#70133=ORIENTED_EDGE('',*,*,#49326,.F.);
#70134=ORIENTED_EDGE('',*,*,#51219,.F.);
#70135=ORIENTED_EDGE('',*,*,#47542,.F.);
#70136=ORIENTED_EDGE('',*,*,#51218,.T.);
#70137=ORIENTED_EDGE('',*,*,#47569,.F.);
#70138=ORIENTED_EDGE('',*,*,#51220,.F.);
#70139=ORIENTED_EDGE('',*,*,#49324,.F.);
#70140=ORIENTED_EDGE('',*,*,#51219,.T.);
#70141=ORIENTED_EDGE('',*,*,#49325,.F.);
#70142=ORIENTED_EDGE('',*,*,#51220,.T.);
#70143=ORIENTED_EDGE('',*,*,#47547,.F.);
#70144=ORIENTED_EDGE('',*,*,#47543,.T.);
#70145=ORIENTED_EDGE('',*,*,#51221,.F.);
#70146=ORIENTED_EDGE('',*,*,#49365,.F.);
#70147=ORIENTED_EDGE('',*,*,#51222,.F.);
#70148=ORIENTED_EDGE('',*,*,#47499,.F.);
#70149=ORIENTED_EDGE('',*,*,#51222,.T.);
#70150=ORIENTED_EDGE('',*,*,#49364,.F.);
#70151=ORIENTED_EDGE('',*,*,#51223,.F.);
#70152=ORIENTED_EDGE('',*,*,#47508,.F.);
#70153=ORIENTED_EDGE('',*,*,#47498,.T.);
#70154=ORIENTED_EDGE('',*,*,#47502,.F.);
#70155=ORIENTED_EDGE('',*,*,#51224,.F.);
#70156=ORIENTED_EDGE('',*,*,#49366,.F.);
#70157=ORIENTED_EDGE('',*,*,#51221,.T.);
#70158=ORIENTED_EDGE('',*,*,#51223,.T.);
#70159=ORIENTED_EDGE('',*,*,#49363,.F.);
#70160=ORIENTED_EDGE('',*,*,#51225,.F.);
#70161=ORIENTED_EDGE('',*,*,#47493,.F.);
#70162=ORIENTED_EDGE('',*,*,#51224,.T.);
#70163=ORIENTED_EDGE('',*,*,#47506,.F.);
#70164=ORIENTED_EDGE('',*,*,#51226,.F.);
#70165=ORIENTED_EDGE('',*,*,#49355,.F.);
#70166=ORIENTED_EDGE('',*,*,#51225,.T.);
#70167=ORIENTED_EDGE('',*,*,#49362,.F.);
#70168=ORIENTED_EDGE('',*,*,#51227,.F.);
#70169=ORIENTED_EDGE('',*,*,#47510,.F.);
#70170=ORIENTED_EDGE('',*,*,#51226,.T.);
#70171=ORIENTED_EDGE('',*,*,#46105,.F.);
#70172=ORIENTED_EDGE('',*,*,#51228,.F.);
#70173=ORIENTED_EDGE('',*,*,#49356,.F.);
#70174=ORIENTED_EDGE('',*,*,#51227,.T.);
#70175=ORIENTED_EDGE('',*,*,#49361,.F.);
#70176=ORIENTED_EDGE('',*,*,#51229,.F.);
#70177=ORIENTED_EDGE('',*,*,#47485,.T.);
#70178=ORIENTED_EDGE('',*,*,#47489,.F.);
#70179=ORIENTED_EDGE('',*,*,#51228,.T.);
#70180=ORIENTED_EDGE('',*,*,#46104,.F.);
#70181=ORIENTED_EDGE('',*,*,#51230,.F.);
#70182=ORIENTED_EDGE('',*,*,#50269,.F.);
#70183=ORIENTED_EDGE('',*,*,#51229,.T.);
#70184=ORIENTED_EDGE('',*,*,#49360,.F.);
#70185=ORIENTED_EDGE('',*,*,#51231,.F.);
#70186=ORIENTED_EDGE('',*,*,#47486,.F.);
#70187=ORIENTED_EDGE('',*,*,#51230,.T.);
#70188=ORIENTED_EDGE('',*,*,#46103,.F.);
#70189=ORIENTED_EDGE('',*,*,#51232,.F.);
#70190=ORIENTED_EDGE('',*,*,#49340,.F.);
#70191=ORIENTED_EDGE('',*,*,#51231,.T.);
#70192=ORIENTED_EDGE('',*,*,#49359,.F.);
#70193=ORIENTED_EDGE('',*,*,#51233,.F.);
#70194=ORIENTED_EDGE('',*,*,#47504,.F.);
#70195=ORIENTED_EDGE('',*,*,#51232,.T.);
#70196=ORIENTED_EDGE('',*,*,#46102,.F.);
#70197=ORIENTED_EDGE('',*,*,#51234,.F.);
#70198=ORIENTED_EDGE('',*,*,#50271,.F.);
#70199=ORIENTED_EDGE('',*,*,#51233,.T.);
#70200=ORIENTED_EDGE('',*,*,#49358,.F.);
#70201=ORIENTED_EDGE('',*,*,#51235,.F.);
#70202=ORIENTED_EDGE('',*,*,#46628,.F.);
#70203=ORIENTED_EDGE('',*,*,#51234,.T.);
#70204=ORIENTED_EDGE('',*,*,#46101,.F.);
#70205=ORIENTED_EDGE('',*,*,#51236,.F.);
#70206=ORIENTED_EDGE('',*,*,#49346,.F.);
#70207=ORIENTED_EDGE('',*,*,#51235,.T.);
#70208=ORIENTED_EDGE('',*,*,#50270,.F.);
#70209=ORIENTED_EDGE('',*,*,#51237,.F.);
#70210=ORIENTED_EDGE('',*,*,#46629,.F.);
#70211=ORIENTED_EDGE('',*,*,#51236,.T.);
#70212=ORIENTED_EDGE('',*,*,#47535,.F.);
#70213=ORIENTED_EDGE('',*,*,#51238,.F.);
#70214=ORIENTED_EDGE('',*,*,#49347,.F.);
#70215=ORIENTED_EDGE('',*,*,#51237,.T.);
#70216=ORIENTED_EDGE('',*,*,#49342,.F.);
#70217=ORIENTED_EDGE('',*,*,#51239,.F.);
#70218=ORIENTED_EDGE('',*,*,#46630,.F.);
#70219=ORIENTED_EDGE('',*,*,#47530,.F.);
#70220=ORIENTED_EDGE('',*,*,#47526,.T.);
#70221=ORIENTED_EDGE('',*,*,#51240,.F.);
#70222=ORIENTED_EDGE('',*,*,#49348,.F.);
#70223=ORIENTED_EDGE('',*,*,#51238,.T.);
#70224=ORIENTED_EDGE('',*,*,#51239,.T.);
#70225=ORIENTED_EDGE('',*,*,#50272,.F.);
#70226=ORIENTED_EDGE('',*,*,#51241,.F.);
#70227=ORIENTED_EDGE('',*,*,#46631,.F.);
#70228=ORIENTED_EDGE('',*,*,#51240,.T.);
#70229=ORIENTED_EDGE('',*,*,#47525,.F.);
#70230=ORIENTED_EDGE('',*,*,#51242,.F.);
#70231=ORIENTED_EDGE('',*,*,#49349,.F.);
#70232=ORIENTED_EDGE('',*,*,#51241,.T.);
#70233=ORIENTED_EDGE('',*,*,#49344,.F.);
#70234=ORIENTED_EDGE('',*,*,#51243,.F.);
#70235=ORIENTED_EDGE('',*,*,#46632,.F.);
#70236=ORIENTED_EDGE('',*,*,#51242,.T.);
#70237=ORIENTED_EDGE('',*,*,#47537,.F.);
#70238=ORIENTED_EDGE('',*,*,#51244,.F.);
#70239=ORIENTED_EDGE('',*,*,#49350,.F.);
#70240=ORIENTED_EDGE('',*,*,#51243,.T.);
#70241=ORIENTED_EDGE('',*,*,#49343,.F.);
#70242=ORIENTED_EDGE('',*,*,#51245,.F.);
#70243=ORIENTED_EDGE('',*,*,#47533,.F.);
#70244=ORIENTED_EDGE('',*,*,#51244,.T.);
#70245=ORIENTED_EDGE('',*,*,#47521,.F.);
#70246=ORIENTED_EDGE('',*,*,#51246,.F.);
#70247=ORIENTED_EDGE('',*,*,#49351,.F.);
#70248=ORIENTED_EDGE('',*,*,#51245,.T.);
#70249=ORIENTED_EDGE('',*,*,#49354,.F.);
#70250=ORIENTED_EDGE('',*,*,#51247,.F.);
#70251=ORIENTED_EDGE('',*,*,#47512,.F.);
#70252=ORIENTED_EDGE('',*,*,#51246,.T.);
#70253=ORIENTED_EDGE('',*,*,#47539,.F.);
#70254=ORIENTED_EDGE('',*,*,#51248,.F.);
#70255=ORIENTED_EDGE('',*,*,#49352,.F.);
#70256=ORIENTED_EDGE('',*,*,#51247,.T.);
#70257=ORIENTED_EDGE('',*,*,#49353,.F.);
#70258=ORIENTED_EDGE('',*,*,#51248,.T.);
#70259=ORIENTED_EDGE('',*,*,#47517,.F.);
#70260=ORIENTED_EDGE('',*,*,#47513,.T.);
#70261=ORIENTED_EDGE('',*,*,#51249,.F.);
#70262=ORIENTED_EDGE('',*,*,#49393,.F.);
#70263=ORIENTED_EDGE('',*,*,#51250,.F.);
#70264=ORIENTED_EDGE('',*,*,#47469,.F.);
#70265=ORIENTED_EDGE('',*,*,#51250,.T.);
#70266=ORIENTED_EDGE('',*,*,#49392,.F.);
#70267=ORIENTED_EDGE('',*,*,#51251,.F.);
#70268=ORIENTED_EDGE('',*,*,#47478,.F.);
#70269=ORIENTED_EDGE('',*,*,#47468,.T.);
#70270=ORIENTED_EDGE('',*,*,#47472,.F.);
#70271=ORIENTED_EDGE('',*,*,#51252,.F.);
#70272=ORIENTED_EDGE('',*,*,#49394,.F.);
#70273=ORIENTED_EDGE('',*,*,#51249,.T.);
#70274=ORIENTED_EDGE('',*,*,#51251,.T.);
#70275=ORIENTED_EDGE('',*,*,#49391,.F.);
#70276=ORIENTED_EDGE('',*,*,#51253,.F.);
#70277=ORIENTED_EDGE('',*,*,#47463,.F.);
#70278=ORIENTED_EDGE('',*,*,#51252,.T.);
#70279=ORIENTED_EDGE('',*,*,#47476,.F.);
#70280=ORIENTED_EDGE('',*,*,#51254,.F.);
#70281=ORIENTED_EDGE('',*,*,#49383,.F.);
#70282=ORIENTED_EDGE('',*,*,#51253,.T.);
#70283=ORIENTED_EDGE('',*,*,#49390,.F.);
#70284=ORIENTED_EDGE('',*,*,#51255,.F.);
#70285=ORIENTED_EDGE('',*,*,#47480,.F.);
#70286=ORIENTED_EDGE('',*,*,#51254,.T.);
#70287=ORIENTED_EDGE('',*,*,#46111,.F.);
#70288=ORIENTED_EDGE('',*,*,#51256,.F.);
#70289=ORIENTED_EDGE('',*,*,#49384,.F.);
#70290=ORIENTED_EDGE('',*,*,#51255,.T.);
#70291=ORIENTED_EDGE('',*,*,#49389,.F.);
#70292=ORIENTED_EDGE('',*,*,#51257,.F.);
#70293=ORIENTED_EDGE('',*,*,#47455,.T.);
#70294=ORIENTED_EDGE('',*,*,#47459,.F.);
#70295=ORIENTED_EDGE('',*,*,#51256,.T.);
#70296=ORIENTED_EDGE('',*,*,#46110,.F.);
#70297=ORIENTED_EDGE('',*,*,#51258,.F.);
#70298=ORIENTED_EDGE('',*,*,#50273,.F.);
#70299=ORIENTED_EDGE('',*,*,#51257,.T.);
#70300=ORIENTED_EDGE('',*,*,#49388,.F.);
#70301=ORIENTED_EDGE('',*,*,#51259,.F.);
#70302=ORIENTED_EDGE('',*,*,#47456,.F.);
#70303=ORIENTED_EDGE('',*,*,#51258,.T.);
#70304=ORIENTED_EDGE('',*,*,#46109,.F.);
#70305=ORIENTED_EDGE('',*,*,#51260,.F.);
#70306=ORIENTED_EDGE('',*,*,#49368,.F.);
#70307=ORIENTED_EDGE('',*,*,#51259,.T.);
#70308=ORIENTED_EDGE('',*,*,#49387,.F.);
#70309=ORIENTED_EDGE('',*,*,#51261,.F.);
#70310=ORIENTED_EDGE('',*,*,#47474,.F.);
#70311=ORIENTED_EDGE('',*,*,#51260,.T.);
#70312=ORIENTED_EDGE('',*,*,#46108,.F.);
#70313=ORIENTED_EDGE('',*,*,#51262,.F.);
#70314=ORIENTED_EDGE('',*,*,#50275,.F.);
#70315=ORIENTED_EDGE('',*,*,#51261,.T.);
#70316=ORIENTED_EDGE('',*,*,#49386,.F.);
#70317=ORIENTED_EDGE('',*,*,#51263,.F.);
#70318=ORIENTED_EDGE('',*,*,#46622,.F.);
#70319=ORIENTED_EDGE('',*,*,#51262,.T.);
#70320=ORIENTED_EDGE('',*,*,#46107,.F.);
#70321=ORIENTED_EDGE('',*,*,#51264,.F.);
#70322=ORIENTED_EDGE('',*,*,#49374,.F.);
#70323=ORIENTED_EDGE('',*,*,#51263,.T.);
#70324=ORIENTED_EDGE('',*,*,#50274,.F.);
#70325=ORIENTED_EDGE('',*,*,#51265,.F.);
#70326=ORIENTED_EDGE('',*,*,#46623,.F.);
#70327=ORIENTED_EDGE('',*,*,#51264,.T.);
#70328=ORIENTED_EDGE('',*,*,#47505,.F.);
#70329=ORIENTED_EDGE('',*,*,#51266,.F.);
#70330=ORIENTED_EDGE('',*,*,#49375,.F.);
#70331=ORIENTED_EDGE('',*,*,#51265,.T.);
#70332=ORIENTED_EDGE('',*,*,#49370,.F.);
#70333=ORIENTED_EDGE('',*,*,#51267,.F.);
#70334=ORIENTED_EDGE('',*,*,#46624,.F.);
#70335=ORIENTED_EDGE('',*,*,#47500,.F.);
#70336=ORIENTED_EDGE('',*,*,#47496,.T.);
#70337=ORIENTED_EDGE('',*,*,#51268,.F.);
#70338=ORIENTED_EDGE('',*,*,#49376,.F.);
#70339=ORIENTED_EDGE('',*,*,#51266,.T.);
#70340=ORIENTED_EDGE('',*,*,#51267,.T.);
#70341=ORIENTED_EDGE('',*,*,#50276,.F.);
#70342=ORIENTED_EDGE('',*,*,#51269,.F.);
#70343=ORIENTED_EDGE('',*,*,#46625,.F.);
#70344=ORIENTED_EDGE('',*,*,#51268,.T.);
#70345=ORIENTED_EDGE('',*,*,#47495,.F.);
#70346=ORIENTED_EDGE('',*,*,#51270,.F.);
#70347=ORIENTED_EDGE('',*,*,#49377,.F.);
#70348=ORIENTED_EDGE('',*,*,#51269,.T.);
#70349=ORIENTED_EDGE('',*,*,#49372,.F.);
#70350=ORIENTED_EDGE('',*,*,#51271,.F.);
#70351=ORIENTED_EDGE('',*,*,#46626,.F.);
#70352=ORIENTED_EDGE('',*,*,#51270,.T.);
#70353=ORIENTED_EDGE('',*,*,#47507,.F.);
#70354=ORIENTED_EDGE('',*,*,#51272,.F.);
#70355=ORIENTED_EDGE('',*,*,#49378,.F.);
#70356=ORIENTED_EDGE('',*,*,#51271,.T.);
#70357=ORIENTED_EDGE('',*,*,#49371,.F.);
#70358=ORIENTED_EDGE('',*,*,#51273,.F.);
#70359=ORIENTED_EDGE('',*,*,#47503,.F.);
#70360=ORIENTED_EDGE('',*,*,#51272,.T.);
#70361=ORIENTED_EDGE('',*,*,#47491,.F.);
#70362=ORIENTED_EDGE('',*,*,#51274,.F.);
#70363=ORIENTED_EDGE('',*,*,#49379,.F.);
#70364=ORIENTED_EDGE('',*,*,#51273,.T.);
#70365=ORIENTED_EDGE('',*,*,#49382,.F.);
#70366=ORIENTED_EDGE('',*,*,#51275,.F.);
#70367=ORIENTED_EDGE('',*,*,#47482,.F.);
#70368=ORIENTED_EDGE('',*,*,#51274,.T.);
#70369=ORIENTED_EDGE('',*,*,#47509,.F.);
#70370=ORIENTED_EDGE('',*,*,#51276,.F.);
#70371=ORIENTED_EDGE('',*,*,#49380,.F.);
#70372=ORIENTED_EDGE('',*,*,#51275,.T.);
#70373=ORIENTED_EDGE('',*,*,#49381,.F.);
#70374=ORIENTED_EDGE('',*,*,#51276,.T.);
#70375=ORIENTED_EDGE('',*,*,#47487,.F.);
#70376=ORIENTED_EDGE('',*,*,#47483,.T.);
#70377=ORIENTED_EDGE('',*,*,#51277,.F.);
#70378=ORIENTED_EDGE('',*,*,#49421,.F.);
#70379=ORIENTED_EDGE('',*,*,#51278,.F.);
#70380=ORIENTED_EDGE('',*,*,#47439,.F.);
#70381=ORIENTED_EDGE('',*,*,#51278,.T.);
#70382=ORIENTED_EDGE('',*,*,#49420,.F.);
#70383=ORIENTED_EDGE('',*,*,#51279,.F.);
#70384=ORIENTED_EDGE('',*,*,#47448,.F.);
#70385=ORIENTED_EDGE('',*,*,#47438,.T.);
#70386=ORIENTED_EDGE('',*,*,#47442,.F.);
#70387=ORIENTED_EDGE('',*,*,#51280,.F.);
#70388=ORIENTED_EDGE('',*,*,#49422,.F.);
#70389=ORIENTED_EDGE('',*,*,#51277,.T.);
#70390=ORIENTED_EDGE('',*,*,#51279,.T.);
#70391=ORIENTED_EDGE('',*,*,#49419,.F.);
#70392=ORIENTED_EDGE('',*,*,#51281,.F.);
#70393=ORIENTED_EDGE('',*,*,#47433,.F.);
#70394=ORIENTED_EDGE('',*,*,#51280,.T.);
#70395=ORIENTED_EDGE('',*,*,#47446,.F.);
#70396=ORIENTED_EDGE('',*,*,#51282,.F.);
#70397=ORIENTED_EDGE('',*,*,#49411,.F.);
#70398=ORIENTED_EDGE('',*,*,#51281,.T.);
#70399=ORIENTED_EDGE('',*,*,#49418,.F.);
#70400=ORIENTED_EDGE('',*,*,#51283,.F.);
#70401=ORIENTED_EDGE('',*,*,#47450,.F.);
#70402=ORIENTED_EDGE('',*,*,#51282,.T.);
#70403=ORIENTED_EDGE('',*,*,#46117,.F.);
#70404=ORIENTED_EDGE('',*,*,#51284,.F.);
#70405=ORIENTED_EDGE('',*,*,#49412,.F.);
#70406=ORIENTED_EDGE('',*,*,#51283,.T.);
#70407=ORIENTED_EDGE('',*,*,#49417,.F.);
#70408=ORIENTED_EDGE('',*,*,#51285,.F.);
#70409=ORIENTED_EDGE('',*,*,#47425,.T.);
#70410=ORIENTED_EDGE('',*,*,#47429,.F.);
#70411=ORIENTED_EDGE('',*,*,#51284,.T.);
#70412=ORIENTED_EDGE('',*,*,#46116,.F.);
#70413=ORIENTED_EDGE('',*,*,#51286,.F.);
#70414=ORIENTED_EDGE('',*,*,#50277,.F.);
#70415=ORIENTED_EDGE('',*,*,#51285,.T.);
#70416=ORIENTED_EDGE('',*,*,#49416,.F.);
#70417=ORIENTED_EDGE('',*,*,#51287,.F.);
#70418=ORIENTED_EDGE('',*,*,#47426,.F.);
#70419=ORIENTED_EDGE('',*,*,#51286,.T.);
#70420=ORIENTED_EDGE('',*,*,#46115,.F.);
#70421=ORIENTED_EDGE('',*,*,#51288,.F.);
#70422=ORIENTED_EDGE('',*,*,#49396,.F.);
#70423=ORIENTED_EDGE('',*,*,#51287,.T.);
#70424=ORIENTED_EDGE('',*,*,#49415,.F.);
#70425=ORIENTED_EDGE('',*,*,#51289,.F.);
#70426=ORIENTED_EDGE('',*,*,#47444,.F.);
#70427=ORIENTED_EDGE('',*,*,#51288,.T.);
#70428=ORIENTED_EDGE('',*,*,#46114,.F.);
#70429=ORIENTED_EDGE('',*,*,#51290,.F.);
#70430=ORIENTED_EDGE('',*,*,#50279,.F.);
#70431=ORIENTED_EDGE('',*,*,#51289,.T.);
#70432=ORIENTED_EDGE('',*,*,#49414,.F.);
#70433=ORIENTED_EDGE('',*,*,#51291,.F.);
#70434=ORIENTED_EDGE('',*,*,#46616,.F.);
#70435=ORIENTED_EDGE('',*,*,#51290,.T.);
#70436=ORIENTED_EDGE('',*,*,#46113,.F.);
#70437=ORIENTED_EDGE('',*,*,#51292,.F.);
#70438=ORIENTED_EDGE('',*,*,#49402,.F.);
#70439=ORIENTED_EDGE('',*,*,#51291,.T.);
#70440=ORIENTED_EDGE('',*,*,#50278,.F.);
#70441=ORIENTED_EDGE('',*,*,#51293,.F.);
#70442=ORIENTED_EDGE('',*,*,#46617,.F.);
#70443=ORIENTED_EDGE('',*,*,#51292,.T.);
#70444=ORIENTED_EDGE('',*,*,#47475,.F.);
#70445=ORIENTED_EDGE('',*,*,#51294,.F.);
#70446=ORIENTED_EDGE('',*,*,#49403,.F.);
#70447=ORIENTED_EDGE('',*,*,#51293,.T.);
#70448=ORIENTED_EDGE('',*,*,#49398,.F.);
#70449=ORIENTED_EDGE('',*,*,#51295,.F.);
#70450=ORIENTED_EDGE('',*,*,#46618,.F.);
#70451=ORIENTED_EDGE('',*,*,#47470,.F.);
#70452=ORIENTED_EDGE('',*,*,#47466,.T.);
#70453=ORIENTED_EDGE('',*,*,#51296,.F.);
#70454=ORIENTED_EDGE('',*,*,#49404,.F.);
#70455=ORIENTED_EDGE('',*,*,#51294,.T.);
#70456=ORIENTED_EDGE('',*,*,#51295,.T.);
#70457=ORIENTED_EDGE('',*,*,#50280,.F.);
#70458=ORIENTED_EDGE('',*,*,#51297,.F.);
#70459=ORIENTED_EDGE('',*,*,#46619,.F.);
#70460=ORIENTED_EDGE('',*,*,#51296,.T.);
#70461=ORIENTED_EDGE('',*,*,#47465,.F.);
#70462=ORIENTED_EDGE('',*,*,#51298,.F.);
#70463=ORIENTED_EDGE('',*,*,#49405,.F.);
#70464=ORIENTED_EDGE('',*,*,#51297,.T.);
#70465=ORIENTED_EDGE('',*,*,#49400,.F.);
#70466=ORIENTED_EDGE('',*,*,#51299,.F.);
#70467=ORIENTED_EDGE('',*,*,#46620,.F.);
#70468=ORIENTED_EDGE('',*,*,#51298,.T.);
#70469=ORIENTED_EDGE('',*,*,#47477,.F.);
#70470=ORIENTED_EDGE('',*,*,#51300,.F.);
#70471=ORIENTED_EDGE('',*,*,#49406,.F.);
#70472=ORIENTED_EDGE('',*,*,#51299,.T.);
#70473=ORIENTED_EDGE('',*,*,#49399,.F.);
#70474=ORIENTED_EDGE('',*,*,#51301,.F.);
#70475=ORIENTED_EDGE('',*,*,#47473,.F.);
#70476=ORIENTED_EDGE('',*,*,#51300,.T.);
#70477=ORIENTED_EDGE('',*,*,#47461,.F.);
#70478=ORIENTED_EDGE('',*,*,#51302,.F.);
#70479=ORIENTED_EDGE('',*,*,#49407,.F.);
#70480=ORIENTED_EDGE('',*,*,#51301,.T.);
#70481=ORIENTED_EDGE('',*,*,#49410,.F.);
#70482=ORIENTED_EDGE('',*,*,#51303,.F.);
#70483=ORIENTED_EDGE('',*,*,#47452,.F.);
#70484=ORIENTED_EDGE('',*,*,#51302,.T.);
#70485=ORIENTED_EDGE('',*,*,#47479,.F.);
#70486=ORIENTED_EDGE('',*,*,#51304,.F.);
#70487=ORIENTED_EDGE('',*,*,#49408,.F.);
#70488=ORIENTED_EDGE('',*,*,#51303,.T.);
#70489=ORIENTED_EDGE('',*,*,#49409,.F.);
#70490=ORIENTED_EDGE('',*,*,#51304,.T.);
#70491=ORIENTED_EDGE('',*,*,#47457,.F.);
#70492=ORIENTED_EDGE('',*,*,#47453,.T.);
#70493=ORIENTED_EDGE('',*,*,#51305,.F.);
#70494=ORIENTED_EDGE('',*,*,#49449,.F.);
#70495=ORIENTED_EDGE('',*,*,#51306,.F.);
#70496=ORIENTED_EDGE('',*,*,#47409,.F.);
#70497=ORIENTED_EDGE('',*,*,#51306,.T.);
#70498=ORIENTED_EDGE('',*,*,#49448,.F.);
#70499=ORIENTED_EDGE('',*,*,#51307,.F.);
#70500=ORIENTED_EDGE('',*,*,#47418,.F.);
#70501=ORIENTED_EDGE('',*,*,#47408,.T.);
#70502=ORIENTED_EDGE('',*,*,#47412,.F.);
#70503=ORIENTED_EDGE('',*,*,#51308,.F.);
#70504=ORIENTED_EDGE('',*,*,#49450,.F.);
#70505=ORIENTED_EDGE('',*,*,#51305,.T.);
#70506=ORIENTED_EDGE('',*,*,#51307,.T.);
#70507=ORIENTED_EDGE('',*,*,#49447,.F.);
#70508=ORIENTED_EDGE('',*,*,#51309,.F.);
#70509=ORIENTED_EDGE('',*,*,#47403,.F.);
#70510=ORIENTED_EDGE('',*,*,#51308,.T.);
#70511=ORIENTED_EDGE('',*,*,#47416,.F.);
#70512=ORIENTED_EDGE('',*,*,#51310,.F.);
#70513=ORIENTED_EDGE('',*,*,#49439,.F.);
#70514=ORIENTED_EDGE('',*,*,#51309,.T.);
#70515=ORIENTED_EDGE('',*,*,#49446,.F.);
#70516=ORIENTED_EDGE('',*,*,#51311,.F.);
#70517=ORIENTED_EDGE('',*,*,#47420,.F.);
#70518=ORIENTED_EDGE('',*,*,#51310,.T.);
#70519=ORIENTED_EDGE('',*,*,#46123,.F.);
#70520=ORIENTED_EDGE('',*,*,#51312,.F.);
#70521=ORIENTED_EDGE('',*,*,#49440,.F.);
#70522=ORIENTED_EDGE('',*,*,#51311,.T.);
#70523=ORIENTED_EDGE('',*,*,#49445,.F.);
#70524=ORIENTED_EDGE('',*,*,#51313,.F.);
#70525=ORIENTED_EDGE('',*,*,#47395,.T.);
#70526=ORIENTED_EDGE('',*,*,#47399,.F.);
#70527=ORIENTED_EDGE('',*,*,#51312,.T.);
#70528=ORIENTED_EDGE('',*,*,#46122,.F.);
#70529=ORIENTED_EDGE('',*,*,#51314,.F.);
#70530=ORIENTED_EDGE('',*,*,#50281,.F.);
#70531=ORIENTED_EDGE('',*,*,#51313,.T.);
#70532=ORIENTED_EDGE('',*,*,#49444,.F.);
#70533=ORIENTED_EDGE('',*,*,#51315,.F.);
#70534=ORIENTED_EDGE('',*,*,#47396,.F.);
#70535=ORIENTED_EDGE('',*,*,#51314,.T.);
#70536=ORIENTED_EDGE('',*,*,#46121,.F.);
#70537=ORIENTED_EDGE('',*,*,#51316,.F.);
#70538=ORIENTED_EDGE('',*,*,#49424,.F.);
#70539=ORIENTED_EDGE('',*,*,#51315,.T.);
#70540=ORIENTED_EDGE('',*,*,#49443,.F.);
#70541=ORIENTED_EDGE('',*,*,#51317,.F.);
#70542=ORIENTED_EDGE('',*,*,#47414,.F.);
#70543=ORIENTED_EDGE('',*,*,#51316,.T.);
#70544=ORIENTED_EDGE('',*,*,#46120,.F.);
#70545=ORIENTED_EDGE('',*,*,#51318,.F.);
#70546=ORIENTED_EDGE('',*,*,#50283,.F.);
#70547=ORIENTED_EDGE('',*,*,#51317,.T.);
#70548=ORIENTED_EDGE('',*,*,#49442,.F.);
#70549=ORIENTED_EDGE('',*,*,#51319,.F.);
#70550=ORIENTED_EDGE('',*,*,#46610,.F.);
#70551=ORIENTED_EDGE('',*,*,#51318,.T.);
#70552=ORIENTED_EDGE('',*,*,#46119,.F.);
#70553=ORIENTED_EDGE('',*,*,#51320,.F.);
#70554=ORIENTED_EDGE('',*,*,#49430,.F.);
#70555=ORIENTED_EDGE('',*,*,#51319,.T.);
#70556=ORIENTED_EDGE('',*,*,#50282,.F.);
#70557=ORIENTED_EDGE('',*,*,#51321,.F.);
#70558=ORIENTED_EDGE('',*,*,#46611,.F.);
#70559=ORIENTED_EDGE('',*,*,#51320,.T.);
#70560=ORIENTED_EDGE('',*,*,#47445,.F.);
#70561=ORIENTED_EDGE('',*,*,#51322,.F.);
#70562=ORIENTED_EDGE('',*,*,#49431,.F.);
#70563=ORIENTED_EDGE('',*,*,#51321,.T.);
#70564=ORIENTED_EDGE('',*,*,#49426,.F.);
#70565=ORIENTED_EDGE('',*,*,#51323,.F.);
#70566=ORIENTED_EDGE('',*,*,#46612,.F.);
#70567=ORIENTED_EDGE('',*,*,#47440,.F.);
#70568=ORIENTED_EDGE('',*,*,#47436,.T.);
#70569=ORIENTED_EDGE('',*,*,#51324,.F.);
#70570=ORIENTED_EDGE('',*,*,#49432,.F.);
#70571=ORIENTED_EDGE('',*,*,#51322,.T.);
#70572=ORIENTED_EDGE('',*,*,#51323,.T.);
#70573=ORIENTED_EDGE('',*,*,#50284,.F.);
#70574=ORIENTED_EDGE('',*,*,#51325,.F.);
#70575=ORIENTED_EDGE('',*,*,#46613,.F.);
#70576=ORIENTED_EDGE('',*,*,#51324,.T.);
#70577=ORIENTED_EDGE('',*,*,#47435,.F.);
#70578=ORIENTED_EDGE('',*,*,#51326,.F.);
#70579=ORIENTED_EDGE('',*,*,#49433,.F.);
#70580=ORIENTED_EDGE('',*,*,#51325,.T.);
#70581=ORIENTED_EDGE('',*,*,#49428,.F.);
#70582=ORIENTED_EDGE('',*,*,#51327,.F.);
#70583=ORIENTED_EDGE('',*,*,#46614,.F.);
#70584=ORIENTED_EDGE('',*,*,#51326,.T.);
#70585=ORIENTED_EDGE('',*,*,#47447,.F.);
#70586=ORIENTED_EDGE('',*,*,#51328,.F.);
#70587=ORIENTED_EDGE('',*,*,#49434,.F.);
#70588=ORIENTED_EDGE('',*,*,#51327,.T.);
#70589=ORIENTED_EDGE('',*,*,#49427,.F.);
#70590=ORIENTED_EDGE('',*,*,#51329,.F.);
#70591=ORIENTED_EDGE('',*,*,#47443,.F.);
#70592=ORIENTED_EDGE('',*,*,#51328,.T.);
#70593=ORIENTED_EDGE('',*,*,#47431,.F.);
#70594=ORIENTED_EDGE('',*,*,#51330,.F.);
#70595=ORIENTED_EDGE('',*,*,#49435,.F.);
#70596=ORIENTED_EDGE('',*,*,#51329,.T.);
#70597=ORIENTED_EDGE('',*,*,#49438,.F.);
#70598=ORIENTED_EDGE('',*,*,#51331,.F.);
#70599=ORIENTED_EDGE('',*,*,#47422,.F.);
#70600=ORIENTED_EDGE('',*,*,#51330,.T.);
#70601=ORIENTED_EDGE('',*,*,#47449,.F.);
#70602=ORIENTED_EDGE('',*,*,#51332,.F.);
#70603=ORIENTED_EDGE('',*,*,#49436,.F.);
#70604=ORIENTED_EDGE('',*,*,#51331,.T.);
#70605=ORIENTED_EDGE('',*,*,#49437,.F.);
#70606=ORIENTED_EDGE('',*,*,#51332,.T.);
#70607=ORIENTED_EDGE('',*,*,#47427,.F.);
#70608=ORIENTED_EDGE('',*,*,#47423,.T.);
#70609=ORIENTED_EDGE('',*,*,#51333,.F.);
#70610=ORIENTED_EDGE('',*,*,#49477,.F.);
#70611=ORIENTED_EDGE('',*,*,#51334,.F.);
#70612=ORIENTED_EDGE('',*,*,#47379,.F.);
#70613=ORIENTED_EDGE('',*,*,#51334,.T.);
#70614=ORIENTED_EDGE('',*,*,#49476,.F.);
#70615=ORIENTED_EDGE('',*,*,#51335,.F.);
#70616=ORIENTED_EDGE('',*,*,#47388,.F.);
#70617=ORIENTED_EDGE('',*,*,#47378,.T.);
#70618=ORIENTED_EDGE('',*,*,#47382,.F.);
#70619=ORIENTED_EDGE('',*,*,#51336,.F.);
#70620=ORIENTED_EDGE('',*,*,#49478,.F.);
#70621=ORIENTED_EDGE('',*,*,#51333,.T.);
#70622=ORIENTED_EDGE('',*,*,#51335,.T.);
#70623=ORIENTED_EDGE('',*,*,#49475,.F.);
#70624=ORIENTED_EDGE('',*,*,#51337,.F.);
#70625=ORIENTED_EDGE('',*,*,#47373,.F.);
#70626=ORIENTED_EDGE('',*,*,#51336,.T.);
#70627=ORIENTED_EDGE('',*,*,#47386,.F.);
#70628=ORIENTED_EDGE('',*,*,#51338,.F.);
#70629=ORIENTED_EDGE('',*,*,#49467,.F.);
#70630=ORIENTED_EDGE('',*,*,#51337,.T.);
#70631=ORIENTED_EDGE('',*,*,#49474,.F.);
#70632=ORIENTED_EDGE('',*,*,#51339,.F.);
#70633=ORIENTED_EDGE('',*,*,#47390,.F.);
#70634=ORIENTED_EDGE('',*,*,#51338,.T.);
#70635=ORIENTED_EDGE('',*,*,#46129,.F.);
#70636=ORIENTED_EDGE('',*,*,#51340,.F.);
#70637=ORIENTED_EDGE('',*,*,#49468,.F.);
#70638=ORIENTED_EDGE('',*,*,#51339,.T.);
#70639=ORIENTED_EDGE('',*,*,#49473,.F.);
#70640=ORIENTED_EDGE('',*,*,#51341,.F.);
#70641=ORIENTED_EDGE('',*,*,#47365,.T.);
#70642=ORIENTED_EDGE('',*,*,#47369,.F.);
#70643=ORIENTED_EDGE('',*,*,#51340,.T.);
#70644=ORIENTED_EDGE('',*,*,#46128,.F.);
#70645=ORIENTED_EDGE('',*,*,#51342,.F.);
#70646=ORIENTED_EDGE('',*,*,#50285,.F.);
#70647=ORIENTED_EDGE('',*,*,#51341,.T.);
#70648=ORIENTED_EDGE('',*,*,#49472,.F.);
#70649=ORIENTED_EDGE('',*,*,#51343,.F.);
#70650=ORIENTED_EDGE('',*,*,#47366,.F.);
#70651=ORIENTED_EDGE('',*,*,#51342,.T.);
#70652=ORIENTED_EDGE('',*,*,#46127,.F.);
#70653=ORIENTED_EDGE('',*,*,#51344,.F.);
#70654=ORIENTED_EDGE('',*,*,#49452,.F.);
#70655=ORIENTED_EDGE('',*,*,#51343,.T.);
#70656=ORIENTED_EDGE('',*,*,#49471,.F.);
#70657=ORIENTED_EDGE('',*,*,#51345,.F.);
#70658=ORIENTED_EDGE('',*,*,#47384,.F.);
#70659=ORIENTED_EDGE('',*,*,#51344,.T.);
#70660=ORIENTED_EDGE('',*,*,#46126,.F.);
#70661=ORIENTED_EDGE('',*,*,#51346,.F.);
#70662=ORIENTED_EDGE('',*,*,#50287,.F.);
#70663=ORIENTED_EDGE('',*,*,#51345,.T.);
#70664=ORIENTED_EDGE('',*,*,#49470,.F.);
#70665=ORIENTED_EDGE('',*,*,#51347,.F.);
#70666=ORIENTED_EDGE('',*,*,#46604,.F.);
#70667=ORIENTED_EDGE('',*,*,#51346,.T.);
#70668=ORIENTED_EDGE('',*,*,#46125,.F.);
#70669=ORIENTED_EDGE('',*,*,#51348,.F.);
#70670=ORIENTED_EDGE('',*,*,#49458,.F.);
#70671=ORIENTED_EDGE('',*,*,#51347,.T.);
#70672=ORIENTED_EDGE('',*,*,#50286,.F.);
#70673=ORIENTED_EDGE('',*,*,#51349,.F.);
#70674=ORIENTED_EDGE('',*,*,#46605,.F.);
#70675=ORIENTED_EDGE('',*,*,#51348,.T.);
#70676=ORIENTED_EDGE('',*,*,#47415,.F.);
#70677=ORIENTED_EDGE('',*,*,#51350,.F.);
#70678=ORIENTED_EDGE('',*,*,#49459,.F.);
#70679=ORIENTED_EDGE('',*,*,#51349,.T.);
#70680=ORIENTED_EDGE('',*,*,#49454,.F.);
#70681=ORIENTED_EDGE('',*,*,#51351,.F.);
#70682=ORIENTED_EDGE('',*,*,#46606,.F.);
#70683=ORIENTED_EDGE('',*,*,#47410,.F.);
#70684=ORIENTED_EDGE('',*,*,#47406,.T.);
#70685=ORIENTED_EDGE('',*,*,#51352,.F.);
#70686=ORIENTED_EDGE('',*,*,#49460,.F.);
#70687=ORIENTED_EDGE('',*,*,#51350,.T.);
#70688=ORIENTED_EDGE('',*,*,#51351,.T.);
#70689=ORIENTED_EDGE('',*,*,#50288,.F.);
#70690=ORIENTED_EDGE('',*,*,#51353,.F.);
#70691=ORIENTED_EDGE('',*,*,#46607,.F.);
#70692=ORIENTED_EDGE('',*,*,#51352,.T.);
#70693=ORIENTED_EDGE('',*,*,#47405,.F.);
#70694=ORIENTED_EDGE('',*,*,#51354,.F.);
#70695=ORIENTED_EDGE('',*,*,#49461,.F.);
#70696=ORIENTED_EDGE('',*,*,#51353,.T.);
#70697=ORIENTED_EDGE('',*,*,#49456,.F.);
#70698=ORIENTED_EDGE('',*,*,#51355,.F.);
#70699=ORIENTED_EDGE('',*,*,#46608,.F.);
#70700=ORIENTED_EDGE('',*,*,#51354,.T.);
#70701=ORIENTED_EDGE('',*,*,#47417,.F.);
#70702=ORIENTED_EDGE('',*,*,#51356,.F.);
#70703=ORIENTED_EDGE('',*,*,#49462,.F.);
#70704=ORIENTED_EDGE('',*,*,#51355,.T.);
#70705=ORIENTED_EDGE('',*,*,#49455,.F.);
#70706=ORIENTED_EDGE('',*,*,#51357,.F.);
#70707=ORIENTED_EDGE('',*,*,#47413,.F.);
#70708=ORIENTED_EDGE('',*,*,#51356,.T.);
#70709=ORIENTED_EDGE('',*,*,#47401,.F.);
#70710=ORIENTED_EDGE('',*,*,#51358,.F.);
#70711=ORIENTED_EDGE('',*,*,#49463,.F.);
#70712=ORIENTED_EDGE('',*,*,#51357,.T.);
#70713=ORIENTED_EDGE('',*,*,#49466,.F.);
#70714=ORIENTED_EDGE('',*,*,#51359,.F.);
#70715=ORIENTED_EDGE('',*,*,#47392,.F.);
#70716=ORIENTED_EDGE('',*,*,#51358,.T.);
#70717=ORIENTED_EDGE('',*,*,#47419,.F.);
#70718=ORIENTED_EDGE('',*,*,#51360,.F.);
#70719=ORIENTED_EDGE('',*,*,#49464,.F.);
#70720=ORIENTED_EDGE('',*,*,#51359,.T.);
#70721=ORIENTED_EDGE('',*,*,#49465,.F.);
#70722=ORIENTED_EDGE('',*,*,#51360,.T.);
#70723=ORIENTED_EDGE('',*,*,#47397,.F.);
#70724=ORIENTED_EDGE('',*,*,#47393,.T.);
#70725=ORIENTED_EDGE('',*,*,#51361,.F.);
#70726=ORIENTED_EDGE('',*,*,#49505,.F.);
#70727=ORIENTED_EDGE('',*,*,#51362,.F.);
#70728=ORIENTED_EDGE('',*,*,#47349,.F.);
#70729=ORIENTED_EDGE('',*,*,#51362,.T.);
#70730=ORIENTED_EDGE('',*,*,#49504,.F.);
#70731=ORIENTED_EDGE('',*,*,#51363,.F.);
#70732=ORIENTED_EDGE('',*,*,#47358,.F.);
#70733=ORIENTED_EDGE('',*,*,#47348,.T.);
#70734=ORIENTED_EDGE('',*,*,#47352,.F.);
#70735=ORIENTED_EDGE('',*,*,#51364,.F.);
#70736=ORIENTED_EDGE('',*,*,#49506,.F.);
#70737=ORIENTED_EDGE('',*,*,#51361,.T.);
#70738=ORIENTED_EDGE('',*,*,#51363,.T.);
#70739=ORIENTED_EDGE('',*,*,#49503,.F.);
#70740=ORIENTED_EDGE('',*,*,#51365,.F.);
#70741=ORIENTED_EDGE('',*,*,#47343,.F.);
#70742=ORIENTED_EDGE('',*,*,#51364,.T.);
#70743=ORIENTED_EDGE('',*,*,#47356,.F.);
#70744=ORIENTED_EDGE('',*,*,#51366,.F.);
#70745=ORIENTED_EDGE('',*,*,#49495,.F.);
#70746=ORIENTED_EDGE('',*,*,#51365,.T.);
#70747=ORIENTED_EDGE('',*,*,#49502,.F.);
#70748=ORIENTED_EDGE('',*,*,#51367,.F.);
#70749=ORIENTED_EDGE('',*,*,#47360,.F.);
#70750=ORIENTED_EDGE('',*,*,#51366,.T.);
#70751=ORIENTED_EDGE('',*,*,#46135,.F.);
#70752=ORIENTED_EDGE('',*,*,#51368,.F.);
#70753=ORIENTED_EDGE('',*,*,#49496,.F.);
#70754=ORIENTED_EDGE('',*,*,#51367,.T.);
#70755=ORIENTED_EDGE('',*,*,#49501,.F.);
#70756=ORIENTED_EDGE('',*,*,#51369,.F.);
#70757=ORIENTED_EDGE('',*,*,#47335,.T.);
#70758=ORIENTED_EDGE('',*,*,#47339,.F.);
#70759=ORIENTED_EDGE('',*,*,#51368,.T.);
#70760=ORIENTED_EDGE('',*,*,#46134,.F.);
#70761=ORIENTED_EDGE('',*,*,#51370,.F.);
#70762=ORIENTED_EDGE('',*,*,#50289,.F.);
#70763=ORIENTED_EDGE('',*,*,#51369,.T.);
#70764=ORIENTED_EDGE('',*,*,#49500,.F.);
#70765=ORIENTED_EDGE('',*,*,#51371,.F.);
#70766=ORIENTED_EDGE('',*,*,#47336,.F.);
#70767=ORIENTED_EDGE('',*,*,#51370,.T.);
#70768=ORIENTED_EDGE('',*,*,#46133,.F.);
#70769=ORIENTED_EDGE('',*,*,#51372,.F.);
#70770=ORIENTED_EDGE('',*,*,#49480,.F.);
#70771=ORIENTED_EDGE('',*,*,#51371,.T.);
#70772=ORIENTED_EDGE('',*,*,#49499,.F.);
#70773=ORIENTED_EDGE('',*,*,#51373,.F.);
#70774=ORIENTED_EDGE('',*,*,#47354,.F.);
#70775=ORIENTED_EDGE('',*,*,#51372,.T.);
#70776=ORIENTED_EDGE('',*,*,#46132,.F.);
#70777=ORIENTED_EDGE('',*,*,#51374,.F.);
#70778=ORIENTED_EDGE('',*,*,#50291,.F.);
#70779=ORIENTED_EDGE('',*,*,#51373,.T.);
#70780=ORIENTED_EDGE('',*,*,#49498,.F.);
#70781=ORIENTED_EDGE('',*,*,#51375,.F.);
#70782=ORIENTED_EDGE('',*,*,#46598,.F.);
#70783=ORIENTED_EDGE('',*,*,#51374,.T.);
#70784=ORIENTED_EDGE('',*,*,#46131,.F.);
#70785=ORIENTED_EDGE('',*,*,#51376,.F.);
#70786=ORIENTED_EDGE('',*,*,#49486,.F.);
#70787=ORIENTED_EDGE('',*,*,#51375,.T.);
#70788=ORIENTED_EDGE('',*,*,#50290,.F.);
#70789=ORIENTED_EDGE('',*,*,#51377,.F.);
#70790=ORIENTED_EDGE('',*,*,#46599,.F.);
#70791=ORIENTED_EDGE('',*,*,#51376,.T.);
#70792=ORIENTED_EDGE('',*,*,#47385,.F.);
#70793=ORIENTED_EDGE('',*,*,#51378,.F.);
#70794=ORIENTED_EDGE('',*,*,#49487,.F.);
#70795=ORIENTED_EDGE('',*,*,#51377,.T.);
#70796=ORIENTED_EDGE('',*,*,#49482,.F.);
#70797=ORIENTED_EDGE('',*,*,#51379,.F.);
#70798=ORIENTED_EDGE('',*,*,#46600,.F.);
#70799=ORIENTED_EDGE('',*,*,#47380,.F.);
#70800=ORIENTED_EDGE('',*,*,#47376,.T.);
#70801=ORIENTED_EDGE('',*,*,#51380,.F.);
#70802=ORIENTED_EDGE('',*,*,#49488,.F.);
#70803=ORIENTED_EDGE('',*,*,#51378,.T.);
#70804=ORIENTED_EDGE('',*,*,#51379,.T.);
#70805=ORIENTED_EDGE('',*,*,#50292,.F.);
#70806=ORIENTED_EDGE('',*,*,#51381,.F.);
#70807=ORIENTED_EDGE('',*,*,#46601,.F.);
#70808=ORIENTED_EDGE('',*,*,#51380,.T.);
#70809=ORIENTED_EDGE('',*,*,#47375,.F.);
#70810=ORIENTED_EDGE('',*,*,#51382,.F.);
#70811=ORIENTED_EDGE('',*,*,#49489,.F.);
#70812=ORIENTED_EDGE('',*,*,#51381,.T.);
#70813=ORIENTED_EDGE('',*,*,#49484,.F.);
#70814=ORIENTED_EDGE('',*,*,#51383,.F.);
#70815=ORIENTED_EDGE('',*,*,#46602,.F.);
#70816=ORIENTED_EDGE('',*,*,#51382,.T.);
#70817=ORIENTED_EDGE('',*,*,#47387,.F.);
#70818=ORIENTED_EDGE('',*,*,#51384,.F.);
#70819=ORIENTED_EDGE('',*,*,#49490,.F.);
#70820=ORIENTED_EDGE('',*,*,#51383,.T.);
#70821=ORIENTED_EDGE('',*,*,#49483,.F.);
#70822=ORIENTED_EDGE('',*,*,#51385,.F.);
#70823=ORIENTED_EDGE('',*,*,#47383,.F.);
#70824=ORIENTED_EDGE('',*,*,#51384,.T.);
#70825=ORIENTED_EDGE('',*,*,#47371,.F.);
#70826=ORIENTED_EDGE('',*,*,#51386,.F.);
#70827=ORIENTED_EDGE('',*,*,#49491,.F.);
#70828=ORIENTED_EDGE('',*,*,#51385,.T.);
#70829=ORIENTED_EDGE('',*,*,#49494,.F.);
#70830=ORIENTED_EDGE('',*,*,#51387,.F.);
#70831=ORIENTED_EDGE('',*,*,#47362,.F.);
#70832=ORIENTED_EDGE('',*,*,#51386,.T.);
#70833=ORIENTED_EDGE('',*,*,#47389,.F.);
#70834=ORIENTED_EDGE('',*,*,#51388,.F.);
#70835=ORIENTED_EDGE('',*,*,#49492,.F.);
#70836=ORIENTED_EDGE('',*,*,#51387,.T.);
#70837=ORIENTED_EDGE('',*,*,#49493,.F.);
#70838=ORIENTED_EDGE('',*,*,#51388,.T.);
#70839=ORIENTED_EDGE('',*,*,#47367,.F.);
#70840=ORIENTED_EDGE('',*,*,#47363,.T.);
#70841=ORIENTED_EDGE('',*,*,#51389,.F.);
#70842=ORIENTED_EDGE('',*,*,#49533,.F.);
#70843=ORIENTED_EDGE('',*,*,#51390,.F.);
#70844=ORIENTED_EDGE('',*,*,#47319,.F.);
#70845=ORIENTED_EDGE('',*,*,#51390,.T.);
#70846=ORIENTED_EDGE('',*,*,#49532,.F.);
#70847=ORIENTED_EDGE('',*,*,#51391,.F.);
#70848=ORIENTED_EDGE('',*,*,#47328,.F.);
#70849=ORIENTED_EDGE('',*,*,#47318,.T.);
#70850=ORIENTED_EDGE('',*,*,#47322,.F.);
#70851=ORIENTED_EDGE('',*,*,#51392,.F.);
#70852=ORIENTED_EDGE('',*,*,#49534,.F.);
#70853=ORIENTED_EDGE('',*,*,#51389,.T.);
#70854=ORIENTED_EDGE('',*,*,#51391,.T.);
#70855=ORIENTED_EDGE('',*,*,#49531,.F.);
#70856=ORIENTED_EDGE('',*,*,#51393,.F.);
#70857=ORIENTED_EDGE('',*,*,#47313,.F.);
#70858=ORIENTED_EDGE('',*,*,#51392,.T.);
#70859=ORIENTED_EDGE('',*,*,#47326,.F.);
#70860=ORIENTED_EDGE('',*,*,#51394,.F.);
#70861=ORIENTED_EDGE('',*,*,#49523,.F.);
#70862=ORIENTED_EDGE('',*,*,#51393,.T.);
#70863=ORIENTED_EDGE('',*,*,#49530,.F.);
#70864=ORIENTED_EDGE('',*,*,#51395,.F.);
#70865=ORIENTED_EDGE('',*,*,#47330,.F.);
#70866=ORIENTED_EDGE('',*,*,#51394,.T.);
#70867=ORIENTED_EDGE('',*,*,#46141,.F.);
#70868=ORIENTED_EDGE('',*,*,#51396,.F.);
#70869=ORIENTED_EDGE('',*,*,#49524,.F.);
#70870=ORIENTED_EDGE('',*,*,#51395,.T.);
#70871=ORIENTED_EDGE('',*,*,#49529,.F.);
#70872=ORIENTED_EDGE('',*,*,#51397,.F.);
#70873=ORIENTED_EDGE('',*,*,#47305,.T.);
#70874=ORIENTED_EDGE('',*,*,#47309,.F.);
#70875=ORIENTED_EDGE('',*,*,#51396,.T.);
#70876=ORIENTED_EDGE('',*,*,#46140,.F.);
#70877=ORIENTED_EDGE('',*,*,#51398,.F.);
#70878=ORIENTED_EDGE('',*,*,#50293,.F.);
#70879=ORIENTED_EDGE('',*,*,#51397,.T.);
#70880=ORIENTED_EDGE('',*,*,#49528,.F.);
#70881=ORIENTED_EDGE('',*,*,#51399,.F.);
#70882=ORIENTED_EDGE('',*,*,#47306,.F.);
#70883=ORIENTED_EDGE('',*,*,#51398,.T.);
#70884=ORIENTED_EDGE('',*,*,#46139,.F.);
#70885=ORIENTED_EDGE('',*,*,#51400,.F.);
#70886=ORIENTED_EDGE('',*,*,#49508,.F.);
#70887=ORIENTED_EDGE('',*,*,#51399,.T.);
#70888=ORIENTED_EDGE('',*,*,#49527,.F.);
#70889=ORIENTED_EDGE('',*,*,#51401,.F.);
#70890=ORIENTED_EDGE('',*,*,#47324,.F.);
#70891=ORIENTED_EDGE('',*,*,#51400,.T.);
#70892=ORIENTED_EDGE('',*,*,#46138,.F.);
#70893=ORIENTED_EDGE('',*,*,#51402,.F.);
#70894=ORIENTED_EDGE('',*,*,#50295,.F.);
#70895=ORIENTED_EDGE('',*,*,#51401,.T.);
#70896=ORIENTED_EDGE('',*,*,#49526,.F.);
#70897=ORIENTED_EDGE('',*,*,#51403,.F.);
#70898=ORIENTED_EDGE('',*,*,#46592,.F.);
#70899=ORIENTED_EDGE('',*,*,#51402,.T.);
#70900=ORIENTED_EDGE('',*,*,#46137,.F.);
#70901=ORIENTED_EDGE('',*,*,#51404,.F.);
#70902=ORIENTED_EDGE('',*,*,#49514,.F.);
#70903=ORIENTED_EDGE('',*,*,#51403,.T.);
#70904=ORIENTED_EDGE('',*,*,#50294,.F.);
#70905=ORIENTED_EDGE('',*,*,#51405,.F.);
#70906=ORIENTED_EDGE('',*,*,#46593,.F.);
#70907=ORIENTED_EDGE('',*,*,#51404,.T.);
#70908=ORIENTED_EDGE('',*,*,#47355,.F.);
#70909=ORIENTED_EDGE('',*,*,#51406,.F.);
#70910=ORIENTED_EDGE('',*,*,#49515,.F.);
#70911=ORIENTED_EDGE('',*,*,#51405,.T.);
#70912=ORIENTED_EDGE('',*,*,#49510,.F.);
#70913=ORIENTED_EDGE('',*,*,#51407,.F.);
#70914=ORIENTED_EDGE('',*,*,#46594,.F.);
#70915=ORIENTED_EDGE('',*,*,#47350,.F.);
#70916=ORIENTED_EDGE('',*,*,#47346,.T.);
#70917=ORIENTED_EDGE('',*,*,#51408,.F.);
#70918=ORIENTED_EDGE('',*,*,#49516,.F.);
#70919=ORIENTED_EDGE('',*,*,#51406,.T.);
#70920=ORIENTED_EDGE('',*,*,#51407,.T.);
#70921=ORIENTED_EDGE('',*,*,#50296,.F.);
#70922=ORIENTED_EDGE('',*,*,#51409,.F.);
#70923=ORIENTED_EDGE('',*,*,#46595,.F.);
#70924=ORIENTED_EDGE('',*,*,#51408,.T.);
#70925=ORIENTED_EDGE('',*,*,#47345,.F.);
#70926=ORIENTED_EDGE('',*,*,#51410,.F.);
#70927=ORIENTED_EDGE('',*,*,#49517,.F.);
#70928=ORIENTED_EDGE('',*,*,#51409,.T.);
#70929=ORIENTED_EDGE('',*,*,#49512,.F.);
#70930=ORIENTED_EDGE('',*,*,#51411,.F.);
#70931=ORIENTED_EDGE('',*,*,#46596,.F.);
#70932=ORIENTED_EDGE('',*,*,#51410,.T.);
#70933=ORIENTED_EDGE('',*,*,#47357,.F.);
#70934=ORIENTED_EDGE('',*,*,#51412,.F.);
#70935=ORIENTED_EDGE('',*,*,#49518,.F.);
#70936=ORIENTED_EDGE('',*,*,#51411,.T.);
#70937=ORIENTED_EDGE('',*,*,#49511,.F.);
#70938=ORIENTED_EDGE('',*,*,#51413,.F.);
#70939=ORIENTED_EDGE('',*,*,#47353,.F.);
#70940=ORIENTED_EDGE('',*,*,#51412,.T.);
#70941=ORIENTED_EDGE('',*,*,#47341,.F.);
#70942=ORIENTED_EDGE('',*,*,#51414,.F.);
#70943=ORIENTED_EDGE('',*,*,#49519,.F.);
#70944=ORIENTED_EDGE('',*,*,#51413,.T.);
#70945=ORIENTED_EDGE('',*,*,#49522,.F.);
#70946=ORIENTED_EDGE('',*,*,#51415,.F.);
#70947=ORIENTED_EDGE('',*,*,#47332,.F.);
#70948=ORIENTED_EDGE('',*,*,#51414,.T.);
#70949=ORIENTED_EDGE('',*,*,#47359,.F.);
#70950=ORIENTED_EDGE('',*,*,#51416,.F.);
#70951=ORIENTED_EDGE('',*,*,#49520,.F.);
#70952=ORIENTED_EDGE('',*,*,#51415,.T.);
#70953=ORIENTED_EDGE('',*,*,#49521,.F.);
#70954=ORIENTED_EDGE('',*,*,#51416,.T.);
#70955=ORIENTED_EDGE('',*,*,#47337,.F.);
#70956=ORIENTED_EDGE('',*,*,#47333,.T.);
#70957=ORIENTED_EDGE('',*,*,#51417,.F.);
#70958=ORIENTED_EDGE('',*,*,#49561,.F.);
#70959=ORIENTED_EDGE('',*,*,#51418,.F.);
#70960=ORIENTED_EDGE('',*,*,#47289,.F.);
#70961=ORIENTED_EDGE('',*,*,#51418,.T.);
#70962=ORIENTED_EDGE('',*,*,#49560,.F.);
#70963=ORIENTED_EDGE('',*,*,#51419,.F.);
#70964=ORIENTED_EDGE('',*,*,#47298,.F.);
#70965=ORIENTED_EDGE('',*,*,#47288,.T.);
#70966=ORIENTED_EDGE('',*,*,#47292,.F.);
#70967=ORIENTED_EDGE('',*,*,#51420,.F.);
#70968=ORIENTED_EDGE('',*,*,#49562,.F.);
#70969=ORIENTED_EDGE('',*,*,#51417,.T.);
#70970=ORIENTED_EDGE('',*,*,#51419,.T.);
#70971=ORIENTED_EDGE('',*,*,#49559,.F.);
#70972=ORIENTED_EDGE('',*,*,#51421,.F.);
#70973=ORIENTED_EDGE('',*,*,#47283,.F.);
#70974=ORIENTED_EDGE('',*,*,#51420,.T.);
#70975=ORIENTED_EDGE('',*,*,#47296,.F.);
#70976=ORIENTED_EDGE('',*,*,#51422,.F.);
#70977=ORIENTED_EDGE('',*,*,#49551,.F.);
#70978=ORIENTED_EDGE('',*,*,#51421,.T.);
#70979=ORIENTED_EDGE('',*,*,#49558,.F.);
#70980=ORIENTED_EDGE('',*,*,#51423,.F.);
#70981=ORIENTED_EDGE('',*,*,#47300,.F.);
#70982=ORIENTED_EDGE('',*,*,#51422,.T.);
#70983=ORIENTED_EDGE('',*,*,#46147,.F.);
#70984=ORIENTED_EDGE('',*,*,#51424,.F.);
#70985=ORIENTED_EDGE('',*,*,#49552,.F.);
#70986=ORIENTED_EDGE('',*,*,#51423,.T.);
#70987=ORIENTED_EDGE('',*,*,#49557,.F.);
#70988=ORIENTED_EDGE('',*,*,#51425,.F.);
#70989=ORIENTED_EDGE('',*,*,#47275,.T.);
#70990=ORIENTED_EDGE('',*,*,#47279,.F.);
#70991=ORIENTED_EDGE('',*,*,#51424,.T.);
#70992=ORIENTED_EDGE('',*,*,#46146,.F.);
#70993=ORIENTED_EDGE('',*,*,#51426,.F.);
#70994=ORIENTED_EDGE('',*,*,#50297,.F.);
#70995=ORIENTED_EDGE('',*,*,#51425,.T.);
#70996=ORIENTED_EDGE('',*,*,#49556,.F.);
#70997=ORIENTED_EDGE('',*,*,#51427,.F.);
#70998=ORIENTED_EDGE('',*,*,#47276,.F.);
#70999=ORIENTED_EDGE('',*,*,#51426,.T.);
#71000=ORIENTED_EDGE('',*,*,#46145,.F.);
#71001=ORIENTED_EDGE('',*,*,#51428,.F.);
#71002=ORIENTED_EDGE('',*,*,#49536,.F.);
#71003=ORIENTED_EDGE('',*,*,#51427,.T.);
#71004=ORIENTED_EDGE('',*,*,#49555,.F.);
#71005=ORIENTED_EDGE('',*,*,#51429,.F.);
#71006=ORIENTED_EDGE('',*,*,#47294,.F.);
#71007=ORIENTED_EDGE('',*,*,#51428,.T.);
#71008=ORIENTED_EDGE('',*,*,#46144,.F.);
#71009=ORIENTED_EDGE('',*,*,#51430,.F.);
#71010=ORIENTED_EDGE('',*,*,#50299,.F.);
#71011=ORIENTED_EDGE('',*,*,#51429,.T.);
#71012=ORIENTED_EDGE('',*,*,#49554,.F.);
#71013=ORIENTED_EDGE('',*,*,#51431,.F.);
#71014=ORIENTED_EDGE('',*,*,#46586,.F.);
#71015=ORIENTED_EDGE('',*,*,#51430,.T.);
#71016=ORIENTED_EDGE('',*,*,#46143,.F.);
#71017=ORIENTED_EDGE('',*,*,#51432,.F.);
#71018=ORIENTED_EDGE('',*,*,#49542,.F.);
#71019=ORIENTED_EDGE('',*,*,#51431,.T.);
#71020=ORIENTED_EDGE('',*,*,#50298,.F.);
#71021=ORIENTED_EDGE('',*,*,#51433,.F.);
#71022=ORIENTED_EDGE('',*,*,#46587,.F.);
#71023=ORIENTED_EDGE('',*,*,#51432,.T.);
#71024=ORIENTED_EDGE('',*,*,#47325,.F.);
#71025=ORIENTED_EDGE('',*,*,#51434,.F.);
#71026=ORIENTED_EDGE('',*,*,#49543,.F.);
#71027=ORIENTED_EDGE('',*,*,#51433,.T.);
#71028=ORIENTED_EDGE('',*,*,#49538,.F.);
#71029=ORIENTED_EDGE('',*,*,#51435,.F.);
#71030=ORIENTED_EDGE('',*,*,#46588,.F.);
#71031=ORIENTED_EDGE('',*,*,#47320,.F.);
#71032=ORIENTED_EDGE('',*,*,#47316,.T.);
#71033=ORIENTED_EDGE('',*,*,#51436,.F.);
#71034=ORIENTED_EDGE('',*,*,#49544,.F.);
#71035=ORIENTED_EDGE('',*,*,#51434,.T.);
#71036=ORIENTED_EDGE('',*,*,#51435,.T.);
#71037=ORIENTED_EDGE('',*,*,#50300,.F.);
#71038=ORIENTED_EDGE('',*,*,#51437,.F.);
#71039=ORIENTED_EDGE('',*,*,#46589,.F.);
#71040=ORIENTED_EDGE('',*,*,#51436,.T.);
#71041=ORIENTED_EDGE('',*,*,#47315,.F.);
#71042=ORIENTED_EDGE('',*,*,#51438,.F.);
#71043=ORIENTED_EDGE('',*,*,#49545,.F.);
#71044=ORIENTED_EDGE('',*,*,#51437,.T.);
#71045=ORIENTED_EDGE('',*,*,#49540,.F.);
#71046=ORIENTED_EDGE('',*,*,#51439,.F.);
#71047=ORIENTED_EDGE('',*,*,#46590,.F.);
#71048=ORIENTED_EDGE('',*,*,#51438,.T.);
#71049=ORIENTED_EDGE('',*,*,#47327,.F.);
#71050=ORIENTED_EDGE('',*,*,#51440,.F.);
#71051=ORIENTED_EDGE('',*,*,#49546,.F.);
#71052=ORIENTED_EDGE('',*,*,#51439,.T.);
#71053=ORIENTED_EDGE('',*,*,#49539,.F.);
#71054=ORIENTED_EDGE('',*,*,#51441,.F.);
#71055=ORIENTED_EDGE('',*,*,#47323,.F.);
#71056=ORIENTED_EDGE('',*,*,#51440,.T.);
#71057=ORIENTED_EDGE('',*,*,#47311,.F.);
#71058=ORIENTED_EDGE('',*,*,#51442,.F.);
#71059=ORIENTED_EDGE('',*,*,#49547,.F.);
#71060=ORIENTED_EDGE('',*,*,#51441,.T.);
#71061=ORIENTED_EDGE('',*,*,#49550,.F.);
#71062=ORIENTED_EDGE('',*,*,#51443,.F.);
#71063=ORIENTED_EDGE('',*,*,#47302,.F.);
#71064=ORIENTED_EDGE('',*,*,#51442,.T.);
#71065=ORIENTED_EDGE('',*,*,#47329,.F.);
#71066=ORIENTED_EDGE('',*,*,#51444,.F.);
#71067=ORIENTED_EDGE('',*,*,#49548,.F.);
#71068=ORIENTED_EDGE('',*,*,#51443,.T.);
#71069=ORIENTED_EDGE('',*,*,#49549,.F.);
#71070=ORIENTED_EDGE('',*,*,#51444,.T.);
#71071=ORIENTED_EDGE('',*,*,#47307,.F.);
#71072=ORIENTED_EDGE('',*,*,#47303,.T.);
#71073=ORIENTED_EDGE('',*,*,#51445,.F.);
#71074=ORIENTED_EDGE('',*,*,#49589,.F.);
#71075=ORIENTED_EDGE('',*,*,#51446,.F.);
#71076=ORIENTED_EDGE('',*,*,#47259,.F.);
#71077=ORIENTED_EDGE('',*,*,#51446,.T.);
#71078=ORIENTED_EDGE('',*,*,#49588,.F.);
#71079=ORIENTED_EDGE('',*,*,#51447,.F.);
#71080=ORIENTED_EDGE('',*,*,#47268,.F.);
#71081=ORIENTED_EDGE('',*,*,#47258,.T.);
#71082=ORIENTED_EDGE('',*,*,#47262,.F.);
#71083=ORIENTED_EDGE('',*,*,#51448,.F.);
#71084=ORIENTED_EDGE('',*,*,#49590,.F.);
#71085=ORIENTED_EDGE('',*,*,#51445,.T.);
#71086=ORIENTED_EDGE('',*,*,#51447,.T.);
#71087=ORIENTED_EDGE('',*,*,#49587,.F.);
#71088=ORIENTED_EDGE('',*,*,#51449,.F.);
#71089=ORIENTED_EDGE('',*,*,#47253,.F.);
#71090=ORIENTED_EDGE('',*,*,#51448,.T.);
#71091=ORIENTED_EDGE('',*,*,#47266,.F.);
#71092=ORIENTED_EDGE('',*,*,#51450,.F.);
#71093=ORIENTED_EDGE('',*,*,#49579,.F.);
#71094=ORIENTED_EDGE('',*,*,#51449,.T.);
#71095=ORIENTED_EDGE('',*,*,#49586,.F.);
#71096=ORIENTED_EDGE('',*,*,#51451,.F.);
#71097=ORIENTED_EDGE('',*,*,#47270,.F.);
#71098=ORIENTED_EDGE('',*,*,#51450,.T.);
#71099=ORIENTED_EDGE('',*,*,#46153,.F.);
#71100=ORIENTED_EDGE('',*,*,#51452,.F.);
#71101=ORIENTED_EDGE('',*,*,#49580,.F.);
#71102=ORIENTED_EDGE('',*,*,#51451,.T.);
#71103=ORIENTED_EDGE('',*,*,#49585,.F.);
#71104=ORIENTED_EDGE('',*,*,#51453,.F.);
#71105=ORIENTED_EDGE('',*,*,#47245,.T.);
#71106=ORIENTED_EDGE('',*,*,#47249,.F.);
#71107=ORIENTED_EDGE('',*,*,#51452,.T.);
#71108=ORIENTED_EDGE('',*,*,#46152,.F.);
#71109=ORIENTED_EDGE('',*,*,#51454,.F.);
#71110=ORIENTED_EDGE('',*,*,#50301,.F.);
#71111=ORIENTED_EDGE('',*,*,#51453,.T.);
#71112=ORIENTED_EDGE('',*,*,#49584,.F.);
#71113=ORIENTED_EDGE('',*,*,#51455,.F.);
#71114=ORIENTED_EDGE('',*,*,#47246,.F.);
#71115=ORIENTED_EDGE('',*,*,#51454,.T.);
#71116=ORIENTED_EDGE('',*,*,#46151,.F.);
#71117=ORIENTED_EDGE('',*,*,#51456,.F.);
#71118=ORIENTED_EDGE('',*,*,#49564,.F.);
#71119=ORIENTED_EDGE('',*,*,#51455,.T.);
#71120=ORIENTED_EDGE('',*,*,#49583,.F.);
#71121=ORIENTED_EDGE('',*,*,#51457,.F.);
#71122=ORIENTED_EDGE('',*,*,#47264,.F.);
#71123=ORIENTED_EDGE('',*,*,#51456,.T.);
#71124=ORIENTED_EDGE('',*,*,#46150,.F.);
#71125=ORIENTED_EDGE('',*,*,#51458,.F.);
#71126=ORIENTED_EDGE('',*,*,#50303,.F.);
#71127=ORIENTED_EDGE('',*,*,#51457,.T.);
#71128=ORIENTED_EDGE('',*,*,#49582,.F.);
#71129=ORIENTED_EDGE('',*,*,#51459,.F.);
#71130=ORIENTED_EDGE('',*,*,#46580,.F.);
#71131=ORIENTED_EDGE('',*,*,#51458,.T.);
#71132=ORIENTED_EDGE('',*,*,#46149,.F.);
#71133=ORIENTED_EDGE('',*,*,#51460,.F.);
#71134=ORIENTED_EDGE('',*,*,#49570,.F.);
#71135=ORIENTED_EDGE('',*,*,#51459,.T.);
#71136=ORIENTED_EDGE('',*,*,#50302,.F.);
#71137=ORIENTED_EDGE('',*,*,#51461,.F.);
#71138=ORIENTED_EDGE('',*,*,#46581,.F.);
#71139=ORIENTED_EDGE('',*,*,#51460,.T.);
#71140=ORIENTED_EDGE('',*,*,#47295,.F.);
#71141=ORIENTED_EDGE('',*,*,#51462,.F.);
#71142=ORIENTED_EDGE('',*,*,#49571,.F.);
#71143=ORIENTED_EDGE('',*,*,#51461,.T.);
#71144=ORIENTED_EDGE('',*,*,#49566,.F.);
#71145=ORIENTED_EDGE('',*,*,#51463,.F.);
#71146=ORIENTED_EDGE('',*,*,#46582,.F.);
#71147=ORIENTED_EDGE('',*,*,#47290,.F.);
#71148=ORIENTED_EDGE('',*,*,#47286,.T.);
#71149=ORIENTED_EDGE('',*,*,#51464,.F.);
#71150=ORIENTED_EDGE('',*,*,#49572,.F.);
#71151=ORIENTED_EDGE('',*,*,#51462,.T.);
#71152=ORIENTED_EDGE('',*,*,#51463,.T.);
#71153=ORIENTED_EDGE('',*,*,#50304,.F.);
#71154=ORIENTED_EDGE('',*,*,#51465,.F.);
#71155=ORIENTED_EDGE('',*,*,#46583,.F.);
#71156=ORIENTED_EDGE('',*,*,#51464,.T.);
#71157=ORIENTED_EDGE('',*,*,#47285,.F.);
#71158=ORIENTED_EDGE('',*,*,#51466,.F.);
#71159=ORIENTED_EDGE('',*,*,#49573,.F.);
#71160=ORIENTED_EDGE('',*,*,#51465,.T.);
#71161=ORIENTED_EDGE('',*,*,#49568,.F.);
#71162=ORIENTED_EDGE('',*,*,#51467,.F.);
#71163=ORIENTED_EDGE('',*,*,#46584,.F.);
#71164=ORIENTED_EDGE('',*,*,#51466,.T.);
#71165=ORIENTED_EDGE('',*,*,#47297,.F.);
#71166=ORIENTED_EDGE('',*,*,#51468,.F.);
#71167=ORIENTED_EDGE('',*,*,#49574,.F.);
#71168=ORIENTED_EDGE('',*,*,#51467,.T.);
#71169=ORIENTED_EDGE('',*,*,#49567,.F.);
#71170=ORIENTED_EDGE('',*,*,#51469,.F.);
#71171=ORIENTED_EDGE('',*,*,#47293,.F.);
#71172=ORIENTED_EDGE('',*,*,#51468,.T.);
#71173=ORIENTED_EDGE('',*,*,#47281,.F.);
#71174=ORIENTED_EDGE('',*,*,#51470,.F.);
#71175=ORIENTED_EDGE('',*,*,#49575,.F.);
#71176=ORIENTED_EDGE('',*,*,#51469,.T.);
#71177=ORIENTED_EDGE('',*,*,#49578,.F.);
#71178=ORIENTED_EDGE('',*,*,#51471,.F.);
#71179=ORIENTED_EDGE('',*,*,#47272,.F.);
#71180=ORIENTED_EDGE('',*,*,#51470,.T.);
#71181=ORIENTED_EDGE('',*,*,#47299,.F.);
#71182=ORIENTED_EDGE('',*,*,#51472,.F.);
#71183=ORIENTED_EDGE('',*,*,#49576,.F.);
#71184=ORIENTED_EDGE('',*,*,#51471,.T.);
#71185=ORIENTED_EDGE('',*,*,#49577,.F.);
#71186=ORIENTED_EDGE('',*,*,#51472,.T.);
#71187=ORIENTED_EDGE('',*,*,#47277,.F.);
#71188=ORIENTED_EDGE('',*,*,#47273,.T.);
#71189=ORIENTED_EDGE('',*,*,#51473,.F.);
#71190=ORIENTED_EDGE('',*,*,#49617,.F.);
#71191=ORIENTED_EDGE('',*,*,#51474,.F.);
#71192=ORIENTED_EDGE('',*,*,#47229,.F.);
#71193=ORIENTED_EDGE('',*,*,#51474,.T.);
#71194=ORIENTED_EDGE('',*,*,#49616,.F.);
#71195=ORIENTED_EDGE('',*,*,#51475,.F.);
#71196=ORIENTED_EDGE('',*,*,#47238,.F.);
#71197=ORIENTED_EDGE('',*,*,#47228,.T.);
#71198=ORIENTED_EDGE('',*,*,#47232,.F.);
#71199=ORIENTED_EDGE('',*,*,#51476,.F.);
#71200=ORIENTED_EDGE('',*,*,#49618,.F.);
#71201=ORIENTED_EDGE('',*,*,#51473,.T.);
#71202=ORIENTED_EDGE('',*,*,#51475,.T.);
#71203=ORIENTED_EDGE('',*,*,#49615,.F.);
#71204=ORIENTED_EDGE('',*,*,#51477,.F.);
#71205=ORIENTED_EDGE('',*,*,#47223,.F.);
#71206=ORIENTED_EDGE('',*,*,#51476,.T.);
#71207=ORIENTED_EDGE('',*,*,#47236,.F.);
#71208=ORIENTED_EDGE('',*,*,#51478,.F.);
#71209=ORIENTED_EDGE('',*,*,#49607,.F.);
#71210=ORIENTED_EDGE('',*,*,#51477,.T.);
#71211=ORIENTED_EDGE('',*,*,#49614,.F.);
#71212=ORIENTED_EDGE('',*,*,#51479,.F.);
#71213=ORIENTED_EDGE('',*,*,#47240,.F.);
#71214=ORIENTED_EDGE('',*,*,#51478,.T.);
#71215=ORIENTED_EDGE('',*,*,#46159,.F.);
#71216=ORIENTED_EDGE('',*,*,#51480,.F.);
#71217=ORIENTED_EDGE('',*,*,#49608,.F.);
#71218=ORIENTED_EDGE('',*,*,#51479,.T.);
#71219=ORIENTED_EDGE('',*,*,#49613,.F.);
#71220=ORIENTED_EDGE('',*,*,#51481,.F.);
#71221=ORIENTED_EDGE('',*,*,#47215,.T.);
#71222=ORIENTED_EDGE('',*,*,#47219,.F.);
#71223=ORIENTED_EDGE('',*,*,#51480,.T.);
#71224=ORIENTED_EDGE('',*,*,#46158,.F.);
#71225=ORIENTED_EDGE('',*,*,#51482,.F.);
#71226=ORIENTED_EDGE('',*,*,#50305,.F.);
#71227=ORIENTED_EDGE('',*,*,#51481,.T.);
#71228=ORIENTED_EDGE('',*,*,#49612,.F.);
#71229=ORIENTED_EDGE('',*,*,#51483,.F.);
#71230=ORIENTED_EDGE('',*,*,#47216,.F.);
#71231=ORIENTED_EDGE('',*,*,#51482,.T.);
#71232=ORIENTED_EDGE('',*,*,#46157,.F.);
#71233=ORIENTED_EDGE('',*,*,#51484,.F.);
#71234=ORIENTED_EDGE('',*,*,#49592,.F.);
#71235=ORIENTED_EDGE('',*,*,#51483,.T.);
#71236=ORIENTED_EDGE('',*,*,#49611,.F.);
#71237=ORIENTED_EDGE('',*,*,#51485,.F.);
#71238=ORIENTED_EDGE('',*,*,#47234,.F.);
#71239=ORIENTED_EDGE('',*,*,#51484,.T.);
#71240=ORIENTED_EDGE('',*,*,#46156,.F.);
#71241=ORIENTED_EDGE('',*,*,#51486,.F.);
#71242=ORIENTED_EDGE('',*,*,#50307,.F.);
#71243=ORIENTED_EDGE('',*,*,#51485,.T.);
#71244=ORIENTED_EDGE('',*,*,#49610,.F.);
#71245=ORIENTED_EDGE('',*,*,#51487,.F.);
#71246=ORIENTED_EDGE('',*,*,#46574,.F.);
#71247=ORIENTED_EDGE('',*,*,#51486,.T.);
#71248=ORIENTED_EDGE('',*,*,#46155,.F.);
#71249=ORIENTED_EDGE('',*,*,#51488,.F.);
#71250=ORIENTED_EDGE('',*,*,#49598,.F.);
#71251=ORIENTED_EDGE('',*,*,#51487,.T.);
#71252=ORIENTED_EDGE('',*,*,#50306,.F.);
#71253=ORIENTED_EDGE('',*,*,#51489,.F.);
#71254=ORIENTED_EDGE('',*,*,#46575,.F.);
#71255=ORIENTED_EDGE('',*,*,#51488,.T.);
#71256=ORIENTED_EDGE('',*,*,#47265,.F.);
#71257=ORIENTED_EDGE('',*,*,#51490,.F.);
#71258=ORIENTED_EDGE('',*,*,#49599,.F.);
#71259=ORIENTED_EDGE('',*,*,#51489,.T.);
#71260=ORIENTED_EDGE('',*,*,#49594,.F.);
#71261=ORIENTED_EDGE('',*,*,#51491,.F.);
#71262=ORIENTED_EDGE('',*,*,#46576,.F.);
#71263=ORIENTED_EDGE('',*,*,#47260,.F.);
#71264=ORIENTED_EDGE('',*,*,#47256,.T.);
#71265=ORIENTED_EDGE('',*,*,#51492,.F.);
#71266=ORIENTED_EDGE('',*,*,#49600,.F.);
#71267=ORIENTED_EDGE('',*,*,#51490,.T.);
#71268=ORIENTED_EDGE('',*,*,#51491,.T.);
#71269=ORIENTED_EDGE('',*,*,#50308,.F.);
#71270=ORIENTED_EDGE('',*,*,#51493,.F.);
#71271=ORIENTED_EDGE('',*,*,#46577,.F.);
#71272=ORIENTED_EDGE('',*,*,#51492,.T.);
#71273=ORIENTED_EDGE('',*,*,#47255,.F.);
#71274=ORIENTED_EDGE('',*,*,#51494,.F.);
#71275=ORIENTED_EDGE('',*,*,#49601,.F.);
#71276=ORIENTED_EDGE('',*,*,#51493,.T.);
#71277=ORIENTED_EDGE('',*,*,#49596,.F.);
#71278=ORIENTED_EDGE('',*,*,#51495,.F.);
#71279=ORIENTED_EDGE('',*,*,#46578,.F.);
#71280=ORIENTED_EDGE('',*,*,#51494,.T.);
#71281=ORIENTED_EDGE('',*,*,#47267,.F.);
#71282=ORIENTED_EDGE('',*,*,#51496,.F.);
#71283=ORIENTED_EDGE('',*,*,#49602,.F.);
#71284=ORIENTED_EDGE('',*,*,#51495,.T.);
#71285=ORIENTED_EDGE('',*,*,#49595,.F.);
#71286=ORIENTED_EDGE('',*,*,#51497,.F.);
#71287=ORIENTED_EDGE('',*,*,#47263,.F.);
#71288=ORIENTED_EDGE('',*,*,#51496,.T.);
#71289=ORIENTED_EDGE('',*,*,#47251,.F.);
#71290=ORIENTED_EDGE('',*,*,#51498,.F.);
#71291=ORIENTED_EDGE('',*,*,#49603,.F.);
#71292=ORIENTED_EDGE('',*,*,#51497,.T.);
#71293=ORIENTED_EDGE('',*,*,#49606,.F.);
#71294=ORIENTED_EDGE('',*,*,#51499,.F.);
#71295=ORIENTED_EDGE('',*,*,#47242,.F.);
#71296=ORIENTED_EDGE('',*,*,#51498,.T.);
#71297=ORIENTED_EDGE('',*,*,#47269,.F.);
#71298=ORIENTED_EDGE('',*,*,#51500,.F.);
#71299=ORIENTED_EDGE('',*,*,#49604,.F.);
#71300=ORIENTED_EDGE('',*,*,#51499,.T.);
#71301=ORIENTED_EDGE('',*,*,#49605,.F.);
#71302=ORIENTED_EDGE('',*,*,#51500,.T.);
#71303=ORIENTED_EDGE('',*,*,#47247,.F.);
#71304=ORIENTED_EDGE('',*,*,#47243,.T.);
#71305=ORIENTED_EDGE('',*,*,#51501,.F.);
#71306=ORIENTED_EDGE('',*,*,#49645,.F.);
#71307=ORIENTED_EDGE('',*,*,#51502,.F.);
#71308=ORIENTED_EDGE('',*,*,#47199,.F.);
#71309=ORIENTED_EDGE('',*,*,#51502,.T.);
#71310=ORIENTED_EDGE('',*,*,#49644,.F.);
#71311=ORIENTED_EDGE('',*,*,#51503,.F.);
#71312=ORIENTED_EDGE('',*,*,#47208,.F.);
#71313=ORIENTED_EDGE('',*,*,#47198,.T.);
#71314=ORIENTED_EDGE('',*,*,#47202,.F.);
#71315=ORIENTED_EDGE('',*,*,#51504,.F.);
#71316=ORIENTED_EDGE('',*,*,#49646,.F.);
#71317=ORIENTED_EDGE('',*,*,#51501,.T.);
#71318=ORIENTED_EDGE('',*,*,#51503,.T.);
#71319=ORIENTED_EDGE('',*,*,#49643,.F.);
#71320=ORIENTED_EDGE('',*,*,#51505,.F.);
#71321=ORIENTED_EDGE('',*,*,#47193,.F.);
#71322=ORIENTED_EDGE('',*,*,#51504,.T.);
#71323=ORIENTED_EDGE('',*,*,#47206,.F.);
#71324=ORIENTED_EDGE('',*,*,#51506,.F.);
#71325=ORIENTED_EDGE('',*,*,#49635,.F.);
#71326=ORIENTED_EDGE('',*,*,#51505,.T.);
#71327=ORIENTED_EDGE('',*,*,#49642,.F.);
#71328=ORIENTED_EDGE('',*,*,#51507,.F.);
#71329=ORIENTED_EDGE('',*,*,#47210,.F.);
#71330=ORIENTED_EDGE('',*,*,#51506,.T.);
#71331=ORIENTED_EDGE('',*,*,#46165,.F.);
#71332=ORIENTED_EDGE('',*,*,#51508,.F.);
#71333=ORIENTED_EDGE('',*,*,#49636,.F.);
#71334=ORIENTED_EDGE('',*,*,#51507,.T.);
#71335=ORIENTED_EDGE('',*,*,#49641,.F.);
#71336=ORIENTED_EDGE('',*,*,#51509,.F.);
#71337=ORIENTED_EDGE('',*,*,#47185,.T.);
#71338=ORIENTED_EDGE('',*,*,#47189,.F.);
#71339=ORIENTED_EDGE('',*,*,#51508,.T.);
#71340=ORIENTED_EDGE('',*,*,#46164,.F.);
#71341=ORIENTED_EDGE('',*,*,#51510,.F.);
#71342=ORIENTED_EDGE('',*,*,#50309,.F.);
#71343=ORIENTED_EDGE('',*,*,#51509,.T.);
#71344=ORIENTED_EDGE('',*,*,#49640,.F.);
#71345=ORIENTED_EDGE('',*,*,#51511,.F.);
#71346=ORIENTED_EDGE('',*,*,#47186,.F.);
#71347=ORIENTED_EDGE('',*,*,#51510,.T.);
#71348=ORIENTED_EDGE('',*,*,#46163,.F.);
#71349=ORIENTED_EDGE('',*,*,#51512,.F.);
#71350=ORIENTED_EDGE('',*,*,#49620,.F.);
#71351=ORIENTED_EDGE('',*,*,#51511,.T.);
#71352=ORIENTED_EDGE('',*,*,#49639,.F.);
#71353=ORIENTED_EDGE('',*,*,#51513,.F.);
#71354=ORIENTED_EDGE('',*,*,#47204,.F.);
#71355=ORIENTED_EDGE('',*,*,#51512,.T.);
#71356=ORIENTED_EDGE('',*,*,#46162,.F.);
#71357=ORIENTED_EDGE('',*,*,#51514,.F.);
#71358=ORIENTED_EDGE('',*,*,#50311,.F.);
#71359=ORIENTED_EDGE('',*,*,#51513,.T.);
#71360=ORIENTED_EDGE('',*,*,#49638,.F.);
#71361=ORIENTED_EDGE('',*,*,#51515,.F.);
#71362=ORIENTED_EDGE('',*,*,#46568,.F.);
#71363=ORIENTED_EDGE('',*,*,#51514,.T.);
#71364=ORIENTED_EDGE('',*,*,#46161,.F.);
#71365=ORIENTED_EDGE('',*,*,#51516,.F.);
#71366=ORIENTED_EDGE('',*,*,#49626,.F.);
#71367=ORIENTED_EDGE('',*,*,#51515,.T.);
#71368=ORIENTED_EDGE('',*,*,#50310,.F.);
#71369=ORIENTED_EDGE('',*,*,#51517,.F.);
#71370=ORIENTED_EDGE('',*,*,#46569,.F.);
#71371=ORIENTED_EDGE('',*,*,#51516,.T.);
#71372=ORIENTED_EDGE('',*,*,#47235,.F.);
#71373=ORIENTED_EDGE('',*,*,#51518,.F.);
#71374=ORIENTED_EDGE('',*,*,#49627,.F.);
#71375=ORIENTED_EDGE('',*,*,#51517,.T.);
#71376=ORIENTED_EDGE('',*,*,#49622,.F.);
#71377=ORIENTED_EDGE('',*,*,#51519,.F.);
#71378=ORIENTED_EDGE('',*,*,#46570,.F.);
#71379=ORIENTED_EDGE('',*,*,#47230,.F.);
#71380=ORIENTED_EDGE('',*,*,#47226,.T.);
#71381=ORIENTED_EDGE('',*,*,#51520,.F.);
#71382=ORIENTED_EDGE('',*,*,#49628,.F.);
#71383=ORIENTED_EDGE('',*,*,#51518,.T.);
#71384=ORIENTED_EDGE('',*,*,#51519,.T.);
#71385=ORIENTED_EDGE('',*,*,#50312,.F.);
#71386=ORIENTED_EDGE('',*,*,#51521,.F.);
#71387=ORIENTED_EDGE('',*,*,#46571,.F.);
#71388=ORIENTED_EDGE('',*,*,#51520,.T.);
#71389=ORIENTED_EDGE('',*,*,#47225,.F.);
#71390=ORIENTED_EDGE('',*,*,#51522,.F.);
#71391=ORIENTED_EDGE('',*,*,#49629,.F.);
#71392=ORIENTED_EDGE('',*,*,#51521,.T.);
#71393=ORIENTED_EDGE('',*,*,#49624,.F.);
#71394=ORIENTED_EDGE('',*,*,#51523,.F.);
#71395=ORIENTED_EDGE('',*,*,#46572,.F.);
#71396=ORIENTED_EDGE('',*,*,#51522,.T.);
#71397=ORIENTED_EDGE('',*,*,#47237,.F.);
#71398=ORIENTED_EDGE('',*,*,#51524,.F.);
#71399=ORIENTED_EDGE('',*,*,#49630,.F.);
#71400=ORIENTED_EDGE('',*,*,#51523,.T.);
#71401=ORIENTED_EDGE('',*,*,#49623,.F.);
#71402=ORIENTED_EDGE('',*,*,#51525,.F.);
#71403=ORIENTED_EDGE('',*,*,#47233,.F.);
#71404=ORIENTED_EDGE('',*,*,#51524,.T.);
#71405=ORIENTED_EDGE('',*,*,#47221,.F.);
#71406=ORIENTED_EDGE('',*,*,#51526,.F.);
#71407=ORIENTED_EDGE('',*,*,#49631,.F.);
#71408=ORIENTED_EDGE('',*,*,#51525,.T.);
#71409=ORIENTED_EDGE('',*,*,#49634,.F.);
#71410=ORIENTED_EDGE('',*,*,#51527,.F.);
#71411=ORIENTED_EDGE('',*,*,#47212,.F.);
#71412=ORIENTED_EDGE('',*,*,#51526,.T.);
#71413=ORIENTED_EDGE('',*,*,#47239,.F.);
#71414=ORIENTED_EDGE('',*,*,#51528,.F.);
#71415=ORIENTED_EDGE('',*,*,#49632,.F.);
#71416=ORIENTED_EDGE('',*,*,#51527,.T.);
#71417=ORIENTED_EDGE('',*,*,#49633,.F.);
#71418=ORIENTED_EDGE('',*,*,#51528,.T.);
#71419=ORIENTED_EDGE('',*,*,#47217,.F.);
#71420=ORIENTED_EDGE('',*,*,#47213,.T.);
#71421=ORIENTED_EDGE('',*,*,#51529,.F.);
#71422=ORIENTED_EDGE('',*,*,#49673,.F.);
#71423=ORIENTED_EDGE('',*,*,#51530,.F.);
#71424=ORIENTED_EDGE('',*,*,#47169,.F.);
#71425=ORIENTED_EDGE('',*,*,#51530,.T.);
#71426=ORIENTED_EDGE('',*,*,#49672,.F.);
#71427=ORIENTED_EDGE('',*,*,#51531,.F.);
#71428=ORIENTED_EDGE('',*,*,#47178,.F.);
#71429=ORIENTED_EDGE('',*,*,#47168,.T.);
#71430=ORIENTED_EDGE('',*,*,#47172,.F.);
#71431=ORIENTED_EDGE('',*,*,#51532,.F.);
#71432=ORIENTED_EDGE('',*,*,#49674,.F.);
#71433=ORIENTED_EDGE('',*,*,#51529,.T.);
#71434=ORIENTED_EDGE('',*,*,#51531,.T.);
#71435=ORIENTED_EDGE('',*,*,#49671,.F.);
#71436=ORIENTED_EDGE('',*,*,#51533,.F.);
#71437=ORIENTED_EDGE('',*,*,#47163,.F.);
#71438=ORIENTED_EDGE('',*,*,#51532,.T.);
#71439=ORIENTED_EDGE('',*,*,#47176,.F.);
#71440=ORIENTED_EDGE('',*,*,#51534,.F.);
#71441=ORIENTED_EDGE('',*,*,#49663,.F.);
#71442=ORIENTED_EDGE('',*,*,#51533,.T.);
#71443=ORIENTED_EDGE('',*,*,#49670,.F.);
#71444=ORIENTED_EDGE('',*,*,#51535,.F.);
#71445=ORIENTED_EDGE('',*,*,#47180,.F.);
#71446=ORIENTED_EDGE('',*,*,#51534,.T.);
#71447=ORIENTED_EDGE('',*,*,#46171,.F.);
#71448=ORIENTED_EDGE('',*,*,#51536,.F.);
#71449=ORIENTED_EDGE('',*,*,#49664,.F.);
#71450=ORIENTED_EDGE('',*,*,#51535,.T.);
#71451=ORIENTED_EDGE('',*,*,#49669,.F.);
#71452=ORIENTED_EDGE('',*,*,#51537,.F.);
#71453=ORIENTED_EDGE('',*,*,#47155,.T.);
#71454=ORIENTED_EDGE('',*,*,#47159,.F.);
#71455=ORIENTED_EDGE('',*,*,#51536,.T.);
#71456=ORIENTED_EDGE('',*,*,#46170,.F.);
#71457=ORIENTED_EDGE('',*,*,#51538,.F.);
#71458=ORIENTED_EDGE('',*,*,#50313,.F.);
#71459=ORIENTED_EDGE('',*,*,#51537,.T.);
#71460=ORIENTED_EDGE('',*,*,#49668,.F.);
#71461=ORIENTED_EDGE('',*,*,#51539,.F.);
#71462=ORIENTED_EDGE('',*,*,#47156,.F.);
#71463=ORIENTED_EDGE('',*,*,#51538,.T.);
#71464=ORIENTED_EDGE('',*,*,#46169,.F.);
#71465=ORIENTED_EDGE('',*,*,#51540,.F.);
#71466=ORIENTED_EDGE('',*,*,#49648,.F.);
#71467=ORIENTED_EDGE('',*,*,#51539,.T.);
#71468=ORIENTED_EDGE('',*,*,#49667,.F.);
#71469=ORIENTED_EDGE('',*,*,#51541,.F.);
#71470=ORIENTED_EDGE('',*,*,#47174,.F.);
#71471=ORIENTED_EDGE('',*,*,#51540,.T.);
#71472=ORIENTED_EDGE('',*,*,#46168,.F.);
#71473=ORIENTED_EDGE('',*,*,#51542,.F.);
#71474=ORIENTED_EDGE('',*,*,#50315,.F.);
#71475=ORIENTED_EDGE('',*,*,#51541,.T.);
#71476=ORIENTED_EDGE('',*,*,#49666,.F.);
#71477=ORIENTED_EDGE('',*,*,#51543,.F.);
#71478=ORIENTED_EDGE('',*,*,#46562,.F.);
#71479=ORIENTED_EDGE('',*,*,#51542,.T.);
#71480=ORIENTED_EDGE('',*,*,#46167,.F.);
#71481=ORIENTED_EDGE('',*,*,#51544,.F.);
#71482=ORIENTED_EDGE('',*,*,#49654,.F.);
#71483=ORIENTED_EDGE('',*,*,#51543,.T.);
#71484=ORIENTED_EDGE('',*,*,#50314,.F.);
#71485=ORIENTED_EDGE('',*,*,#51545,.F.);
#71486=ORIENTED_EDGE('',*,*,#46563,.F.);
#71487=ORIENTED_EDGE('',*,*,#51544,.T.);
#71488=ORIENTED_EDGE('',*,*,#47205,.F.);
#71489=ORIENTED_EDGE('',*,*,#51546,.F.);
#71490=ORIENTED_EDGE('',*,*,#49655,.F.);
#71491=ORIENTED_EDGE('',*,*,#51545,.T.);
#71492=ORIENTED_EDGE('',*,*,#49650,.F.);
#71493=ORIENTED_EDGE('',*,*,#51547,.F.);
#71494=ORIENTED_EDGE('',*,*,#46564,.F.);
#71495=ORIENTED_EDGE('',*,*,#47200,.F.);
#71496=ORIENTED_EDGE('',*,*,#47196,.T.);
#71497=ORIENTED_EDGE('',*,*,#51548,.F.);
#71498=ORIENTED_EDGE('',*,*,#49656,.F.);
#71499=ORIENTED_EDGE('',*,*,#51546,.T.);
#71500=ORIENTED_EDGE('',*,*,#51547,.T.);
#71501=ORIENTED_EDGE('',*,*,#50316,.F.);
#71502=ORIENTED_EDGE('',*,*,#51549,.F.);
#71503=ORIENTED_EDGE('',*,*,#46565,.F.);
#71504=ORIENTED_EDGE('',*,*,#51548,.T.);
#71505=ORIENTED_EDGE('',*,*,#47195,.F.);
#71506=ORIENTED_EDGE('',*,*,#51550,.F.);
#71507=ORIENTED_EDGE('',*,*,#49657,.F.);
#71508=ORIENTED_EDGE('',*,*,#51549,.T.);
#71509=ORIENTED_EDGE('',*,*,#49652,.F.);
#71510=ORIENTED_EDGE('',*,*,#51551,.F.);
#71511=ORIENTED_EDGE('',*,*,#46566,.F.);
#71512=ORIENTED_EDGE('',*,*,#51550,.T.);
#71513=ORIENTED_EDGE('',*,*,#47207,.F.);
#71514=ORIENTED_EDGE('',*,*,#51552,.F.);
#71515=ORIENTED_EDGE('',*,*,#49658,.F.);
#71516=ORIENTED_EDGE('',*,*,#51551,.T.);
#71517=ORIENTED_EDGE('',*,*,#49651,.F.);
#71518=ORIENTED_EDGE('',*,*,#51553,.F.);
#71519=ORIENTED_EDGE('',*,*,#47203,.F.);
#71520=ORIENTED_EDGE('',*,*,#51552,.T.);
#71521=ORIENTED_EDGE('',*,*,#47191,.F.);
#71522=ORIENTED_EDGE('',*,*,#51554,.F.);
#71523=ORIENTED_EDGE('',*,*,#49659,.F.);
#71524=ORIENTED_EDGE('',*,*,#51553,.T.);
#71525=ORIENTED_EDGE('',*,*,#49662,.F.);
#71526=ORIENTED_EDGE('',*,*,#51555,.F.);
#71527=ORIENTED_EDGE('',*,*,#47182,.F.);
#71528=ORIENTED_EDGE('',*,*,#51554,.T.);
#71529=ORIENTED_EDGE('',*,*,#47209,.F.);
#71530=ORIENTED_EDGE('',*,*,#51556,.F.);
#71531=ORIENTED_EDGE('',*,*,#49660,.F.);
#71532=ORIENTED_EDGE('',*,*,#51555,.T.);
#71533=ORIENTED_EDGE('',*,*,#49661,.F.);
#71534=ORIENTED_EDGE('',*,*,#51556,.T.);
#71535=ORIENTED_EDGE('',*,*,#47187,.F.);
#71536=ORIENTED_EDGE('',*,*,#47183,.T.);
#71537=ORIENTED_EDGE('',*,*,#51557,.F.);
#71538=ORIENTED_EDGE('',*,*,#49701,.F.);
#71539=ORIENTED_EDGE('',*,*,#51558,.F.);
#71540=ORIENTED_EDGE('',*,*,#47139,.F.);
#71541=ORIENTED_EDGE('',*,*,#51558,.T.);
#71542=ORIENTED_EDGE('',*,*,#49700,.F.);
#71543=ORIENTED_EDGE('',*,*,#51559,.F.);
#71544=ORIENTED_EDGE('',*,*,#47148,.F.);
#71545=ORIENTED_EDGE('',*,*,#47138,.T.);
#71546=ORIENTED_EDGE('',*,*,#47142,.F.);
#71547=ORIENTED_EDGE('',*,*,#51560,.F.);
#71548=ORIENTED_EDGE('',*,*,#49702,.F.);
#71549=ORIENTED_EDGE('',*,*,#51557,.T.);
#71550=ORIENTED_EDGE('',*,*,#51559,.T.);
#71551=ORIENTED_EDGE('',*,*,#49699,.F.);
#71552=ORIENTED_EDGE('',*,*,#51561,.F.);
#71553=ORIENTED_EDGE('',*,*,#47133,.F.);
#71554=ORIENTED_EDGE('',*,*,#51560,.T.);
#71555=ORIENTED_EDGE('',*,*,#47146,.F.);
#71556=ORIENTED_EDGE('',*,*,#51562,.F.);
#71557=ORIENTED_EDGE('',*,*,#49691,.F.);
#71558=ORIENTED_EDGE('',*,*,#51561,.T.);
#71559=ORIENTED_EDGE('',*,*,#49698,.F.);
#71560=ORIENTED_EDGE('',*,*,#51563,.F.);
#71561=ORIENTED_EDGE('',*,*,#47150,.F.);
#71562=ORIENTED_EDGE('',*,*,#51562,.T.);
#71563=ORIENTED_EDGE('',*,*,#46177,.F.);
#71564=ORIENTED_EDGE('',*,*,#51564,.F.);
#71565=ORIENTED_EDGE('',*,*,#49692,.F.);
#71566=ORIENTED_EDGE('',*,*,#51563,.T.);
#71567=ORIENTED_EDGE('',*,*,#49697,.F.);
#71568=ORIENTED_EDGE('',*,*,#51565,.F.);
#71569=ORIENTED_EDGE('',*,*,#47125,.T.);
#71570=ORIENTED_EDGE('',*,*,#47129,.F.);
#71571=ORIENTED_EDGE('',*,*,#51564,.T.);
#71572=ORIENTED_EDGE('',*,*,#46176,.F.);
#71573=ORIENTED_EDGE('',*,*,#51566,.F.);
#71574=ORIENTED_EDGE('',*,*,#50317,.F.);
#71575=ORIENTED_EDGE('',*,*,#51565,.T.);
#71576=ORIENTED_EDGE('',*,*,#49696,.F.);
#71577=ORIENTED_EDGE('',*,*,#51567,.F.);
#71578=ORIENTED_EDGE('',*,*,#47126,.F.);
#71579=ORIENTED_EDGE('',*,*,#51566,.T.);
#71580=ORIENTED_EDGE('',*,*,#46175,.F.);
#71581=ORIENTED_EDGE('',*,*,#51568,.F.);
#71582=ORIENTED_EDGE('',*,*,#49676,.F.);
#71583=ORIENTED_EDGE('',*,*,#51567,.T.);
#71584=ORIENTED_EDGE('',*,*,#49695,.F.);
#71585=ORIENTED_EDGE('',*,*,#51569,.F.);
#71586=ORIENTED_EDGE('',*,*,#47144,.F.);
#71587=ORIENTED_EDGE('',*,*,#51568,.T.);
#71588=ORIENTED_EDGE('',*,*,#46174,.F.);
#71589=ORIENTED_EDGE('',*,*,#51570,.F.);
#71590=ORIENTED_EDGE('',*,*,#50319,.F.);
#71591=ORIENTED_EDGE('',*,*,#51569,.T.);
#71592=ORIENTED_EDGE('',*,*,#49694,.F.);
#71593=ORIENTED_EDGE('',*,*,#51571,.F.);
#71594=ORIENTED_EDGE('',*,*,#46556,.F.);
#71595=ORIENTED_EDGE('',*,*,#51570,.T.);
#71596=ORIENTED_EDGE('',*,*,#46173,.F.);
#71597=ORIENTED_EDGE('',*,*,#51572,.F.);
#71598=ORIENTED_EDGE('',*,*,#49682,.F.);
#71599=ORIENTED_EDGE('',*,*,#51571,.T.);
#71600=ORIENTED_EDGE('',*,*,#50318,.F.);
#71601=ORIENTED_EDGE('',*,*,#51573,.F.);
#71602=ORIENTED_EDGE('',*,*,#46557,.F.);
#71603=ORIENTED_EDGE('',*,*,#51572,.T.);
#71604=ORIENTED_EDGE('',*,*,#47175,.F.);
#71605=ORIENTED_EDGE('',*,*,#51574,.F.);
#71606=ORIENTED_EDGE('',*,*,#49683,.F.);
#71607=ORIENTED_EDGE('',*,*,#51573,.T.);
#71608=ORIENTED_EDGE('',*,*,#49678,.F.);
#71609=ORIENTED_EDGE('',*,*,#51575,.F.);
#71610=ORIENTED_EDGE('',*,*,#46558,.F.);
#71611=ORIENTED_EDGE('',*,*,#47170,.F.);
#71612=ORIENTED_EDGE('',*,*,#47166,.T.);
#71613=ORIENTED_EDGE('',*,*,#51576,.F.);
#71614=ORIENTED_EDGE('',*,*,#49684,.F.);
#71615=ORIENTED_EDGE('',*,*,#51574,.T.);
#71616=ORIENTED_EDGE('',*,*,#51575,.T.);
#71617=ORIENTED_EDGE('',*,*,#50320,.F.);
#71618=ORIENTED_EDGE('',*,*,#51577,.F.);
#71619=ORIENTED_EDGE('',*,*,#46559,.F.);
#71620=ORIENTED_EDGE('',*,*,#51576,.T.);
#71621=ORIENTED_EDGE('',*,*,#47165,.F.);
#71622=ORIENTED_EDGE('',*,*,#51578,.F.);
#71623=ORIENTED_EDGE('',*,*,#49685,.F.);
#71624=ORIENTED_EDGE('',*,*,#51577,.T.);
#71625=ORIENTED_EDGE('',*,*,#49680,.F.);
#71626=ORIENTED_EDGE('',*,*,#51579,.F.);
#71627=ORIENTED_EDGE('',*,*,#46560,.F.);
#71628=ORIENTED_EDGE('',*,*,#51578,.T.);
#71629=ORIENTED_EDGE('',*,*,#47177,.F.);
#71630=ORIENTED_EDGE('',*,*,#51580,.F.);
#71631=ORIENTED_EDGE('',*,*,#49686,.F.);
#71632=ORIENTED_EDGE('',*,*,#51579,.T.);
#71633=ORIENTED_EDGE('',*,*,#49679,.F.);
#71634=ORIENTED_EDGE('',*,*,#51581,.F.);
#71635=ORIENTED_EDGE('',*,*,#47173,.F.);
#71636=ORIENTED_EDGE('',*,*,#51580,.T.);
#71637=ORIENTED_EDGE('',*,*,#47161,.F.);
#71638=ORIENTED_EDGE('',*,*,#51582,.F.);
#71639=ORIENTED_EDGE('',*,*,#49687,.F.);
#71640=ORIENTED_EDGE('',*,*,#51581,.T.);
#71641=ORIENTED_EDGE('',*,*,#49690,.F.);
#71642=ORIENTED_EDGE('',*,*,#51583,.F.);
#71643=ORIENTED_EDGE('',*,*,#47152,.F.);
#71644=ORIENTED_EDGE('',*,*,#51582,.T.);
#71645=ORIENTED_EDGE('',*,*,#47179,.F.);
#71646=ORIENTED_EDGE('',*,*,#51584,.F.);
#71647=ORIENTED_EDGE('',*,*,#49688,.F.);
#71648=ORIENTED_EDGE('',*,*,#51583,.T.);
#71649=ORIENTED_EDGE('',*,*,#49689,.F.);
#71650=ORIENTED_EDGE('',*,*,#51584,.T.);
#71651=ORIENTED_EDGE('',*,*,#47157,.F.);
#71652=ORIENTED_EDGE('',*,*,#47153,.T.);
#71653=ORIENTED_EDGE('',*,*,#51585,.F.);
#71654=ORIENTED_EDGE('',*,*,#49729,.F.);
#71655=ORIENTED_EDGE('',*,*,#51586,.F.);
#71656=ORIENTED_EDGE('',*,*,#47109,.F.);
#71657=ORIENTED_EDGE('',*,*,#51586,.T.);
#71658=ORIENTED_EDGE('',*,*,#49728,.F.);
#71659=ORIENTED_EDGE('',*,*,#51587,.F.);
#71660=ORIENTED_EDGE('',*,*,#47118,.F.);
#71661=ORIENTED_EDGE('',*,*,#47108,.T.);
#71662=ORIENTED_EDGE('',*,*,#47112,.F.);
#71663=ORIENTED_EDGE('',*,*,#51588,.F.);
#71664=ORIENTED_EDGE('',*,*,#49730,.F.);
#71665=ORIENTED_EDGE('',*,*,#51585,.T.);
#71666=ORIENTED_EDGE('',*,*,#51587,.T.);
#71667=ORIENTED_EDGE('',*,*,#49727,.F.);
#71668=ORIENTED_EDGE('',*,*,#51589,.F.);
#71669=ORIENTED_EDGE('',*,*,#47103,.F.);
#71670=ORIENTED_EDGE('',*,*,#51588,.T.);
#71671=ORIENTED_EDGE('',*,*,#47116,.F.);
#71672=ORIENTED_EDGE('',*,*,#51590,.F.);
#71673=ORIENTED_EDGE('',*,*,#49719,.F.);
#71674=ORIENTED_EDGE('',*,*,#51589,.T.);
#71675=ORIENTED_EDGE('',*,*,#49726,.F.);
#71676=ORIENTED_EDGE('',*,*,#51591,.F.);
#71677=ORIENTED_EDGE('',*,*,#47120,.F.);
#71678=ORIENTED_EDGE('',*,*,#51590,.T.);
#71679=ORIENTED_EDGE('',*,*,#46183,.F.);
#71680=ORIENTED_EDGE('',*,*,#51592,.F.);
#71681=ORIENTED_EDGE('',*,*,#49720,.F.);
#71682=ORIENTED_EDGE('',*,*,#51591,.T.);
#71683=ORIENTED_EDGE('',*,*,#49725,.F.);
#71684=ORIENTED_EDGE('',*,*,#51593,.F.);
#71685=ORIENTED_EDGE('',*,*,#47095,.T.);
#71686=ORIENTED_EDGE('',*,*,#47099,.F.);
#71687=ORIENTED_EDGE('',*,*,#51592,.T.);
#71688=ORIENTED_EDGE('',*,*,#46182,.F.);
#71689=ORIENTED_EDGE('',*,*,#51594,.F.);
#71690=ORIENTED_EDGE('',*,*,#50321,.F.);
#71691=ORIENTED_EDGE('',*,*,#51593,.T.);
#71692=ORIENTED_EDGE('',*,*,#49724,.F.);
#71693=ORIENTED_EDGE('',*,*,#51595,.F.);
#71694=ORIENTED_EDGE('',*,*,#47096,.F.);
#71695=ORIENTED_EDGE('',*,*,#51594,.T.);
#71696=ORIENTED_EDGE('',*,*,#46181,.F.);
#71697=ORIENTED_EDGE('',*,*,#51596,.F.);
#71698=ORIENTED_EDGE('',*,*,#49704,.F.);
#71699=ORIENTED_EDGE('',*,*,#51595,.T.);
#71700=ORIENTED_EDGE('',*,*,#49723,.F.);
#71701=ORIENTED_EDGE('',*,*,#51597,.F.);
#71702=ORIENTED_EDGE('',*,*,#47114,.F.);
#71703=ORIENTED_EDGE('',*,*,#51596,.T.);
#71704=ORIENTED_EDGE('',*,*,#46180,.F.);
#71705=ORIENTED_EDGE('',*,*,#51598,.F.);
#71706=ORIENTED_EDGE('',*,*,#50323,.F.);
#71707=ORIENTED_EDGE('',*,*,#51597,.T.);
#71708=ORIENTED_EDGE('',*,*,#49722,.F.);
#71709=ORIENTED_EDGE('',*,*,#51599,.F.);
#71710=ORIENTED_EDGE('',*,*,#46550,.F.);
#71711=ORIENTED_EDGE('',*,*,#51598,.T.);
#71712=ORIENTED_EDGE('',*,*,#46179,.F.);
#71713=ORIENTED_EDGE('',*,*,#51600,.F.);
#71714=ORIENTED_EDGE('',*,*,#49710,.F.);
#71715=ORIENTED_EDGE('',*,*,#51599,.T.);
#71716=ORIENTED_EDGE('',*,*,#50322,.F.);
#71717=ORIENTED_EDGE('',*,*,#51601,.F.);
#71718=ORIENTED_EDGE('',*,*,#46551,.F.);
#71719=ORIENTED_EDGE('',*,*,#51600,.T.);
#71720=ORIENTED_EDGE('',*,*,#47145,.F.);
#71721=ORIENTED_EDGE('',*,*,#51602,.F.);
#71722=ORIENTED_EDGE('',*,*,#49711,.F.);
#71723=ORIENTED_EDGE('',*,*,#51601,.T.);
#71724=ORIENTED_EDGE('',*,*,#49706,.F.);
#71725=ORIENTED_EDGE('',*,*,#51603,.F.);
#71726=ORIENTED_EDGE('',*,*,#46552,.F.);
#71727=ORIENTED_EDGE('',*,*,#47140,.F.);
#71728=ORIENTED_EDGE('',*,*,#47136,.T.);
#71729=ORIENTED_EDGE('',*,*,#51604,.F.);
#71730=ORIENTED_EDGE('',*,*,#49712,.F.);
#71731=ORIENTED_EDGE('',*,*,#51602,.T.);
#71732=ORIENTED_EDGE('',*,*,#51603,.T.);
#71733=ORIENTED_EDGE('',*,*,#50324,.F.);
#71734=ORIENTED_EDGE('',*,*,#51605,.F.);
#71735=ORIENTED_EDGE('',*,*,#46553,.F.);
#71736=ORIENTED_EDGE('',*,*,#51604,.T.);
#71737=ORIENTED_EDGE('',*,*,#47135,.F.);
#71738=ORIENTED_EDGE('',*,*,#51606,.F.);
#71739=ORIENTED_EDGE('',*,*,#49713,.F.);
#71740=ORIENTED_EDGE('',*,*,#51605,.T.);
#71741=ORIENTED_EDGE('',*,*,#49708,.F.);
#71742=ORIENTED_EDGE('',*,*,#51607,.F.);
#71743=ORIENTED_EDGE('',*,*,#46554,.F.);
#71744=ORIENTED_EDGE('',*,*,#51606,.T.);
#71745=ORIENTED_EDGE('',*,*,#47147,.F.);
#71746=ORIENTED_EDGE('',*,*,#51608,.F.);
#71747=ORIENTED_EDGE('',*,*,#49714,.F.);
#71748=ORIENTED_EDGE('',*,*,#51607,.T.);
#71749=ORIENTED_EDGE('',*,*,#49707,.F.);
#71750=ORIENTED_EDGE('',*,*,#51609,.F.);
#71751=ORIENTED_EDGE('',*,*,#47143,.F.);
#71752=ORIENTED_EDGE('',*,*,#51608,.T.);
#71753=ORIENTED_EDGE('',*,*,#47131,.F.);
#71754=ORIENTED_EDGE('',*,*,#51610,.F.);
#71755=ORIENTED_EDGE('',*,*,#49715,.F.);
#71756=ORIENTED_EDGE('',*,*,#51609,.T.);
#71757=ORIENTED_EDGE('',*,*,#49718,.F.);
#71758=ORIENTED_EDGE('',*,*,#51611,.F.);
#71759=ORIENTED_EDGE('',*,*,#47122,.F.);
#71760=ORIENTED_EDGE('',*,*,#51610,.T.);
#71761=ORIENTED_EDGE('',*,*,#47149,.F.);
#71762=ORIENTED_EDGE('',*,*,#51612,.F.);
#71763=ORIENTED_EDGE('',*,*,#49716,.F.);
#71764=ORIENTED_EDGE('',*,*,#51611,.T.);
#71765=ORIENTED_EDGE('',*,*,#49717,.F.);
#71766=ORIENTED_EDGE('',*,*,#51612,.T.);
#71767=ORIENTED_EDGE('',*,*,#47127,.F.);
#71768=ORIENTED_EDGE('',*,*,#47123,.T.);
#71769=ORIENTED_EDGE('',*,*,#51613,.F.);
#71770=ORIENTED_EDGE('',*,*,#49755,.F.);
#71771=ORIENTED_EDGE('',*,*,#51614,.F.);
#71772=ORIENTED_EDGE('',*,*,#47079,.F.);
#71773=ORIENTED_EDGE('',*,*,#51614,.T.);
#71774=ORIENTED_EDGE('',*,*,#49754,.F.);
#71775=ORIENTED_EDGE('',*,*,#51615,.F.);
#71776=ORIENTED_EDGE('',*,*,#47088,.F.);
#71777=ORIENTED_EDGE('',*,*,#47078,.T.);
#71778=ORIENTED_EDGE('',*,*,#47082,.F.);
#71779=ORIENTED_EDGE('',*,*,#51616,.F.);
#71780=ORIENTED_EDGE('',*,*,#49756,.F.);
#71781=ORIENTED_EDGE('',*,*,#51613,.T.);
#71782=ORIENTED_EDGE('',*,*,#51615,.T.);
#71783=ORIENTED_EDGE('',*,*,#49753,.F.);
#71784=ORIENTED_EDGE('',*,*,#51617,.F.);
#71785=ORIENTED_EDGE('',*,*,#47073,.F.);
#71786=ORIENTED_EDGE('',*,*,#51616,.T.);
#71787=ORIENTED_EDGE('',*,*,#47086,.F.);
#71788=ORIENTED_EDGE('',*,*,#51618,.F.);
#71789=ORIENTED_EDGE('',*,*,#49745,.F.);
#71790=ORIENTED_EDGE('',*,*,#51617,.T.);
#71791=ORIENTED_EDGE('',*,*,#49752,.F.);
#71792=ORIENTED_EDGE('',*,*,#51619,.F.);
#71793=ORIENTED_EDGE('',*,*,#47090,.F.);
#71794=ORIENTED_EDGE('',*,*,#51618,.T.);
#71795=ORIENTED_EDGE('',*,*,#46188,.F.);
#71796=ORIENTED_EDGE('',*,*,#51620,.F.);
#71797=ORIENTED_EDGE('',*,*,#49746,.F.);
#71798=ORIENTED_EDGE('',*,*,#51619,.T.);
#71799=ORIENTED_EDGE('',*,*,#49751,.F.);
#71800=ORIENTED_EDGE('',*,*,#51621,.F.);
#71801=ORIENTED_EDGE('',*,*,#47065,.T.);
#71802=ORIENTED_EDGE('',*,*,#47069,.F.);
#71803=ORIENTED_EDGE('',*,*,#51620,.T.);
#71804=ORIENTED_EDGE('',*,*,#46187,.F.);
#71805=ORIENTED_EDGE('',*,*,#45889,.F.);
#71806=ORIENTED_EDGE('',*,*,#50325,.F.);
#71807=ORIENTED_EDGE('',*,*,#51621,.T.);
#71808=ORIENTED_EDGE('',*,*,#49750,.F.);
#71809=ORIENTED_EDGE('',*,*,#51622,.F.);
#71810=ORIENTED_EDGE('',*,*,#47066,.F.);
#71811=ORIENTED_EDGE('',*,*,#51622,.T.);
#71812=ORIENTED_EDGE('',*,*,#49749,.F.);
#71813=ORIENTED_EDGE('',*,*,#51623,.F.);
#71814=ORIENTED_EDGE('',*,*,#47084,.F.);
#71815=ORIENTED_EDGE('',*,*,#45887,.T.);
#71816=ORIENTED_EDGE('',*,*,#46186,.F.);
#71817=ORIENTED_EDGE('',*,*,#51624,.F.);
#71818=ORIENTED_EDGE('',*,*,#50327,.F.);
#71819=ORIENTED_EDGE('',*,*,#51623,.T.);
#71820=ORIENTED_EDGE('',*,*,#49748,.F.);
#71821=ORIENTED_EDGE('',*,*,#51625,.F.);
#71822=ORIENTED_EDGE('',*,*,#46545,.F.);
#71823=ORIENTED_EDGE('',*,*,#51624,.T.);
#71824=ORIENTED_EDGE('',*,*,#46185,.F.);
#71825=ORIENTED_EDGE('',*,*,#51626,.F.);
#71826=ORIENTED_EDGE('',*,*,#49736,.F.);
#71827=ORIENTED_EDGE('',*,*,#51625,.T.);
#71828=ORIENTED_EDGE('',*,*,#50326,.F.);
#71829=ORIENTED_EDGE('',*,*,#45885,.F.);
#71830=ORIENTED_EDGE('',*,*,#46546,.F.);
#71831=ORIENTED_EDGE('',*,*,#51626,.T.);
#71832=ORIENTED_EDGE('',*,*,#47115,.F.);
#71833=ORIENTED_EDGE('',*,*,#51627,.F.);
#71834=ORIENTED_EDGE('',*,*,#49737,.F.);
#71835=ORIENTED_EDGE('',*,*,#47110,.F.);
#71836=ORIENTED_EDGE('',*,*,#47106,.T.);
#71837=ORIENTED_EDGE('',*,*,#51628,.F.);
#71838=ORIENTED_EDGE('',*,*,#49738,.F.);
#71839=ORIENTED_EDGE('',*,*,#51627,.T.);
#71840=ORIENTED_EDGE('',*,*,#45883,.T.);
#71841=ORIENTED_EDGE('',*,*,#50328,.F.);
#71842=ORIENTED_EDGE('',*,*,#51629,.F.);
#71843=ORIENTED_EDGE('',*,*,#46547,.F.);
#71844=ORIENTED_EDGE('',*,*,#51628,.T.);
#71845=ORIENTED_EDGE('',*,*,#47105,.F.);
#71846=ORIENTED_EDGE('',*,*,#51630,.F.);
#71847=ORIENTED_EDGE('',*,*,#49739,.F.);
#71848=ORIENTED_EDGE('',*,*,#51629,.T.);
#71849=ORIENTED_EDGE('',*,*,#49734,.F.);
#71850=ORIENTED_EDGE('',*,*,#51631,.F.);
#71851=ORIENTED_EDGE('',*,*,#46548,.F.);
#71852=ORIENTED_EDGE('',*,*,#51630,.T.);
#71853=ORIENTED_EDGE('',*,*,#47117,.F.);
#71854=ORIENTED_EDGE('',*,*,#51632,.F.);
#71855=ORIENTED_EDGE('',*,*,#49740,.F.);
#71856=ORIENTED_EDGE('',*,*,#51631,.T.);
#71857=ORIENTED_EDGE('',*,*,#49733,.F.);
#71858=ORIENTED_EDGE('',*,*,#51633,.F.);
#71859=ORIENTED_EDGE('',*,*,#47113,.F.);
#71860=ORIENTED_EDGE('',*,*,#51632,.T.);
#71861=ORIENTED_EDGE('',*,*,#47101,.F.);
#71862=ORIENTED_EDGE('',*,*,#51634,.F.);
#71863=ORIENTED_EDGE('',*,*,#49741,.F.);
#71864=ORIENTED_EDGE('',*,*,#51633,.T.);
#71865=ORIENTED_EDGE('',*,*,#49744,.F.);
#71866=ORIENTED_EDGE('',*,*,#51635,.F.);
#71867=ORIENTED_EDGE('',*,*,#47092,.F.);
#71868=ORIENTED_EDGE('',*,*,#51634,.T.);
#71869=ORIENTED_EDGE('',*,*,#47119,.F.);
#71870=ORIENTED_EDGE('',*,*,#51636,.F.);
#71871=ORIENTED_EDGE('',*,*,#49742,.F.);
#71872=ORIENTED_EDGE('',*,*,#51635,.T.);
#71873=ORIENTED_EDGE('',*,*,#49743,.F.);
#71874=ORIENTED_EDGE('',*,*,#51636,.T.);
#71875=ORIENTED_EDGE('',*,*,#47097,.F.);
#71876=ORIENTED_EDGE('',*,*,#47093,.T.);
#71877=ORIENTED_EDGE('',*,*,#51637,.F.);
#71878=ORIENTED_EDGE('',*,*,#49783,.F.);
#71879=ORIENTED_EDGE('',*,*,#51638,.F.);
#71880=ORIENTED_EDGE('',*,*,#47049,.F.);
#71881=ORIENTED_EDGE('',*,*,#51638,.T.);
#71882=ORIENTED_EDGE('',*,*,#49782,.F.);
#71883=ORIENTED_EDGE('',*,*,#51639,.F.);
#71884=ORIENTED_EDGE('',*,*,#47058,.F.);
#71885=ORIENTED_EDGE('',*,*,#47048,.T.);
#71886=ORIENTED_EDGE('',*,*,#47052,.F.);
#71887=ORIENTED_EDGE('',*,*,#51640,.F.);
#71888=ORIENTED_EDGE('',*,*,#49784,.F.);
#71889=ORIENTED_EDGE('',*,*,#51637,.T.);
#71890=ORIENTED_EDGE('',*,*,#51639,.T.);
#71891=ORIENTED_EDGE('',*,*,#49781,.F.);
#71892=ORIENTED_EDGE('',*,*,#51641,.F.);
#71893=ORIENTED_EDGE('',*,*,#47043,.F.);
#71894=ORIENTED_EDGE('',*,*,#51640,.T.);
#71895=ORIENTED_EDGE('',*,*,#47056,.F.);
#71896=ORIENTED_EDGE('',*,*,#51642,.F.);
#71897=ORIENTED_EDGE('',*,*,#49773,.F.);
#71898=ORIENTED_EDGE('',*,*,#51641,.T.);
#71899=ORIENTED_EDGE('',*,*,#49780,.F.);
#71900=ORIENTED_EDGE('',*,*,#51643,.F.);
#71901=ORIENTED_EDGE('',*,*,#47060,.F.);
#71902=ORIENTED_EDGE('',*,*,#51642,.T.);
#71903=ORIENTED_EDGE('',*,*,#46194,.F.);
#71904=ORIENTED_EDGE('',*,*,#51644,.F.);
#71905=ORIENTED_EDGE('',*,*,#49774,.F.);
#71906=ORIENTED_EDGE('',*,*,#51643,.T.);
#71907=ORIENTED_EDGE('',*,*,#49779,.F.);
#71908=ORIENTED_EDGE('',*,*,#51645,.F.);
#71909=ORIENTED_EDGE('',*,*,#47035,.T.);
#71910=ORIENTED_EDGE('',*,*,#47039,.F.);
#71911=ORIENTED_EDGE('',*,*,#51644,.T.);
#71912=ORIENTED_EDGE('',*,*,#46193,.F.);
#71913=ORIENTED_EDGE('',*,*,#51646,.F.);
#71914=ORIENTED_EDGE('',*,*,#50329,.F.);
#71915=ORIENTED_EDGE('',*,*,#51645,.T.);
#71916=ORIENTED_EDGE('',*,*,#49778,.F.);
#71917=ORIENTED_EDGE('',*,*,#51647,.F.);
#71918=ORIENTED_EDGE('',*,*,#47036,.F.);
#71919=ORIENTED_EDGE('',*,*,#51646,.T.);
#71920=ORIENTED_EDGE('',*,*,#46192,.F.);
#71921=ORIENTED_EDGE('',*,*,#51648,.F.);
#71922=ORIENTED_EDGE('',*,*,#49758,.F.);
#71923=ORIENTED_EDGE('',*,*,#51647,.T.);
#71924=ORIENTED_EDGE('',*,*,#49777,.F.);
#71925=ORIENTED_EDGE('',*,*,#51649,.F.);
#71926=ORIENTED_EDGE('',*,*,#47054,.F.);
#71927=ORIENTED_EDGE('',*,*,#51648,.T.);
#71928=ORIENTED_EDGE('',*,*,#46191,.F.);
#71929=ORIENTED_EDGE('',*,*,#51650,.F.);
#71930=ORIENTED_EDGE('',*,*,#50331,.F.);
#71931=ORIENTED_EDGE('',*,*,#51649,.T.);
#71932=ORIENTED_EDGE('',*,*,#49776,.F.);
#71933=ORIENTED_EDGE('',*,*,#51651,.F.);
#71934=ORIENTED_EDGE('',*,*,#46539,.F.);
#71935=ORIENTED_EDGE('',*,*,#51650,.T.);
#71936=ORIENTED_EDGE('',*,*,#46190,.F.);
#71937=ORIENTED_EDGE('',*,*,#51652,.F.);
#71938=ORIENTED_EDGE('',*,*,#49764,.F.);
#71939=ORIENTED_EDGE('',*,*,#51651,.T.);
#71940=ORIENTED_EDGE('',*,*,#50330,.F.);
#71941=ORIENTED_EDGE('',*,*,#51653,.F.);
#71942=ORIENTED_EDGE('',*,*,#46540,.F.);
#71943=ORIENTED_EDGE('',*,*,#51652,.T.);
#71944=ORIENTED_EDGE('',*,*,#47085,.F.);
#71945=ORIENTED_EDGE('',*,*,#51654,.F.);
#71946=ORIENTED_EDGE('',*,*,#49765,.F.);
#71947=ORIENTED_EDGE('',*,*,#51653,.T.);
#71948=ORIENTED_EDGE('',*,*,#49760,.F.);
#71949=ORIENTED_EDGE('',*,*,#51655,.F.);
#71950=ORIENTED_EDGE('',*,*,#46541,.F.);
#71951=ORIENTED_EDGE('',*,*,#47080,.F.);
#71952=ORIENTED_EDGE('',*,*,#47076,.T.);
#71953=ORIENTED_EDGE('',*,*,#51656,.F.);
#71954=ORIENTED_EDGE('',*,*,#49766,.F.);
#71955=ORIENTED_EDGE('',*,*,#51654,.T.);
#71956=ORIENTED_EDGE('',*,*,#51655,.T.);
#71957=ORIENTED_EDGE('',*,*,#50332,.F.);
#71958=ORIENTED_EDGE('',*,*,#51657,.F.);
#71959=ORIENTED_EDGE('',*,*,#46542,.F.);
#71960=ORIENTED_EDGE('',*,*,#51656,.T.);
#71961=ORIENTED_EDGE('',*,*,#47075,.F.);
#71962=ORIENTED_EDGE('',*,*,#51658,.F.);
#71963=ORIENTED_EDGE('',*,*,#49767,.F.);
#71964=ORIENTED_EDGE('',*,*,#51657,.T.);
#71965=ORIENTED_EDGE('',*,*,#49762,.F.);
#71966=ORIENTED_EDGE('',*,*,#51659,.F.);
#71967=ORIENTED_EDGE('',*,*,#46543,.F.);
#71968=ORIENTED_EDGE('',*,*,#51658,.T.);
#71969=ORIENTED_EDGE('',*,*,#47087,.F.);
#71970=ORIENTED_EDGE('',*,*,#51660,.F.);
#71971=ORIENTED_EDGE('',*,*,#49768,.F.);
#71972=ORIENTED_EDGE('',*,*,#51659,.T.);
#71973=ORIENTED_EDGE('',*,*,#49761,.F.);
#71974=ORIENTED_EDGE('',*,*,#51661,.F.);
#71975=ORIENTED_EDGE('',*,*,#47083,.F.);
#71976=ORIENTED_EDGE('',*,*,#51660,.T.);
#71977=ORIENTED_EDGE('',*,*,#47071,.F.);
#71978=ORIENTED_EDGE('',*,*,#51662,.F.);
#71979=ORIENTED_EDGE('',*,*,#49769,.F.);
#71980=ORIENTED_EDGE('',*,*,#51661,.T.);
#71981=ORIENTED_EDGE('',*,*,#49772,.F.);
#71982=ORIENTED_EDGE('',*,*,#51663,.F.);
#71983=ORIENTED_EDGE('',*,*,#47062,.F.);
#71984=ORIENTED_EDGE('',*,*,#51662,.T.);
#71985=ORIENTED_EDGE('',*,*,#47089,.F.);
#71986=ORIENTED_EDGE('',*,*,#51664,.F.);
#71987=ORIENTED_EDGE('',*,*,#49770,.F.);
#71988=ORIENTED_EDGE('',*,*,#51663,.T.);
#71989=ORIENTED_EDGE('',*,*,#49771,.F.);
#71990=ORIENTED_EDGE('',*,*,#51664,.T.);
#71991=ORIENTED_EDGE('',*,*,#47067,.F.);
#71992=ORIENTED_EDGE('',*,*,#47063,.T.);
#71993=ORIENTED_EDGE('',*,*,#51665,.F.);
#71994=ORIENTED_EDGE('',*,*,#49811,.F.);
#71995=ORIENTED_EDGE('',*,*,#51666,.F.);
#71996=ORIENTED_EDGE('',*,*,#47019,.F.);
#71997=ORIENTED_EDGE('',*,*,#51666,.T.);
#71998=ORIENTED_EDGE('',*,*,#49810,.F.);
#71999=ORIENTED_EDGE('',*,*,#51667,.F.);
#72000=ORIENTED_EDGE('',*,*,#47028,.F.);
#72001=ORIENTED_EDGE('',*,*,#47018,.T.);
#72002=ORIENTED_EDGE('',*,*,#47022,.F.);
#72003=ORIENTED_EDGE('',*,*,#51668,.F.);
#72004=ORIENTED_EDGE('',*,*,#49812,.F.);
#72005=ORIENTED_EDGE('',*,*,#51665,.T.);
#72006=ORIENTED_EDGE('',*,*,#51667,.T.);
#72007=ORIENTED_EDGE('',*,*,#49809,.F.);
#72008=ORIENTED_EDGE('',*,*,#51669,.F.);
#72009=ORIENTED_EDGE('',*,*,#47013,.F.);
#72010=ORIENTED_EDGE('',*,*,#51668,.T.);
#72011=ORIENTED_EDGE('',*,*,#47026,.F.);
#72012=ORIENTED_EDGE('',*,*,#51670,.F.);
#72013=ORIENTED_EDGE('',*,*,#49801,.F.);
#72014=ORIENTED_EDGE('',*,*,#51669,.T.);
#72015=ORIENTED_EDGE('',*,*,#49808,.F.);
#72016=ORIENTED_EDGE('',*,*,#51671,.F.);
#72017=ORIENTED_EDGE('',*,*,#47030,.F.);
#72018=ORIENTED_EDGE('',*,*,#51670,.T.);
#72019=ORIENTED_EDGE('',*,*,#46200,.F.);
#72020=ORIENTED_EDGE('',*,*,#51672,.F.);
#72021=ORIENTED_EDGE('',*,*,#49802,.F.);
#72022=ORIENTED_EDGE('',*,*,#51671,.T.);
#72023=ORIENTED_EDGE('',*,*,#49807,.F.);
#72024=ORIENTED_EDGE('',*,*,#51673,.F.);
#72025=ORIENTED_EDGE('',*,*,#47005,.T.);
#72026=ORIENTED_EDGE('',*,*,#47009,.F.);
#72027=ORIENTED_EDGE('',*,*,#51672,.T.);
#72028=ORIENTED_EDGE('',*,*,#46199,.F.);
#72029=ORIENTED_EDGE('',*,*,#51674,.F.);
#72030=ORIENTED_EDGE('',*,*,#50333,.F.);
#72031=ORIENTED_EDGE('',*,*,#51673,.T.);
#72032=ORIENTED_EDGE('',*,*,#49806,.F.);
#72033=ORIENTED_EDGE('',*,*,#51675,.F.);
#72034=ORIENTED_EDGE('',*,*,#47006,.F.);
#72035=ORIENTED_EDGE('',*,*,#51674,.T.);
#72036=ORIENTED_EDGE('',*,*,#46198,.F.);
#72037=ORIENTED_EDGE('',*,*,#51676,.F.);
#72038=ORIENTED_EDGE('',*,*,#49786,.F.);
#72039=ORIENTED_EDGE('',*,*,#51675,.T.);
#72040=ORIENTED_EDGE('',*,*,#49805,.F.);
#72041=ORIENTED_EDGE('',*,*,#51677,.F.);
#72042=ORIENTED_EDGE('',*,*,#47024,.F.);
#72043=ORIENTED_EDGE('',*,*,#51676,.T.);
#72044=ORIENTED_EDGE('',*,*,#46197,.F.);
#72045=ORIENTED_EDGE('',*,*,#51678,.F.);
#72046=ORIENTED_EDGE('',*,*,#50335,.F.);
#72047=ORIENTED_EDGE('',*,*,#51677,.T.);
#72048=ORIENTED_EDGE('',*,*,#49804,.F.);
#72049=ORIENTED_EDGE('',*,*,#51679,.F.);
#72050=ORIENTED_EDGE('',*,*,#46533,.F.);
#72051=ORIENTED_EDGE('',*,*,#51678,.T.);
#72052=ORIENTED_EDGE('',*,*,#46196,.F.);
#72053=ORIENTED_EDGE('',*,*,#51680,.F.);
#72054=ORIENTED_EDGE('',*,*,#49792,.F.);
#72055=ORIENTED_EDGE('',*,*,#51679,.T.);
#72056=ORIENTED_EDGE('',*,*,#50334,.F.);
#72057=ORIENTED_EDGE('',*,*,#51681,.F.);
#72058=ORIENTED_EDGE('',*,*,#46534,.F.);
#72059=ORIENTED_EDGE('',*,*,#51680,.T.);
#72060=ORIENTED_EDGE('',*,*,#47055,.F.);
#72061=ORIENTED_EDGE('',*,*,#51682,.F.);
#72062=ORIENTED_EDGE('',*,*,#49793,.F.);
#72063=ORIENTED_EDGE('',*,*,#51681,.T.);
#72064=ORIENTED_EDGE('',*,*,#49788,.F.);
#72065=ORIENTED_EDGE('',*,*,#51683,.F.);
#72066=ORIENTED_EDGE('',*,*,#46535,.F.);
#72067=ORIENTED_EDGE('',*,*,#47050,.F.);
#72068=ORIENTED_EDGE('',*,*,#47046,.T.);
#72069=ORIENTED_EDGE('',*,*,#51684,.F.);
#72070=ORIENTED_EDGE('',*,*,#49794,.F.);
#72071=ORIENTED_EDGE('',*,*,#51682,.T.);
#72072=ORIENTED_EDGE('',*,*,#51683,.T.);
#72073=ORIENTED_EDGE('',*,*,#50336,.F.);
#72074=ORIENTED_EDGE('',*,*,#51685,.F.);
#72075=ORIENTED_EDGE('',*,*,#46536,.F.);
#72076=ORIENTED_EDGE('',*,*,#51684,.T.);
#72077=ORIENTED_EDGE('',*,*,#47045,.F.);
#72078=ORIENTED_EDGE('',*,*,#51686,.F.);
#72079=ORIENTED_EDGE('',*,*,#49795,.F.);
#72080=ORIENTED_EDGE('',*,*,#51685,.T.);
#72081=ORIENTED_EDGE('',*,*,#49790,.F.);
#72082=ORIENTED_EDGE('',*,*,#51687,.F.);
#72083=ORIENTED_EDGE('',*,*,#46537,.F.);
#72084=ORIENTED_EDGE('',*,*,#51686,.T.);
#72085=ORIENTED_EDGE('',*,*,#47057,.F.);
#72086=ORIENTED_EDGE('',*,*,#51688,.F.);
#72087=ORIENTED_EDGE('',*,*,#49796,.F.);
#72088=ORIENTED_EDGE('',*,*,#51687,.T.);
#72089=ORIENTED_EDGE('',*,*,#49789,.F.);
#72090=ORIENTED_EDGE('',*,*,#51689,.F.);
#72091=ORIENTED_EDGE('',*,*,#47053,.F.);
#72092=ORIENTED_EDGE('',*,*,#51688,.T.);
#72093=ORIENTED_EDGE('',*,*,#47041,.F.);
#72094=ORIENTED_EDGE('',*,*,#51690,.F.);
#72095=ORIENTED_EDGE('',*,*,#49797,.F.);
#72096=ORIENTED_EDGE('',*,*,#51689,.T.);
#72097=ORIENTED_EDGE('',*,*,#49800,.F.);
#72098=ORIENTED_EDGE('',*,*,#51691,.F.);
#72099=ORIENTED_EDGE('',*,*,#47032,.F.);
#72100=ORIENTED_EDGE('',*,*,#51690,.T.);
#72101=ORIENTED_EDGE('',*,*,#47059,.F.);
#72102=ORIENTED_EDGE('',*,*,#51692,.F.);
#72103=ORIENTED_EDGE('',*,*,#49798,.F.);
#72104=ORIENTED_EDGE('',*,*,#51691,.T.);
#72105=ORIENTED_EDGE('',*,*,#49799,.F.);
#72106=ORIENTED_EDGE('',*,*,#51692,.T.);
#72107=ORIENTED_EDGE('',*,*,#47037,.F.);
#72108=ORIENTED_EDGE('',*,*,#47033,.T.);
#72109=ORIENTED_EDGE('',*,*,#51693,.F.);
#72110=ORIENTED_EDGE('',*,*,#49839,.F.);
#72111=ORIENTED_EDGE('',*,*,#51694,.F.);
#72112=ORIENTED_EDGE('',*,*,#46989,.F.);
#72113=ORIENTED_EDGE('',*,*,#51694,.T.);
#72114=ORIENTED_EDGE('',*,*,#49838,.F.);
#72115=ORIENTED_EDGE('',*,*,#51695,.F.);
#72116=ORIENTED_EDGE('',*,*,#46998,.F.);
#72117=ORIENTED_EDGE('',*,*,#46988,.T.);
#72118=ORIENTED_EDGE('',*,*,#46992,.F.);
#72119=ORIENTED_EDGE('',*,*,#51696,.F.);
#72120=ORIENTED_EDGE('',*,*,#49840,.F.);
#72121=ORIENTED_EDGE('',*,*,#51693,.T.);
#72122=ORIENTED_EDGE('',*,*,#51695,.T.);
#72123=ORIENTED_EDGE('',*,*,#49837,.F.);
#72124=ORIENTED_EDGE('',*,*,#51697,.F.);
#72125=ORIENTED_EDGE('',*,*,#46983,.F.);
#72126=ORIENTED_EDGE('',*,*,#51696,.T.);
#72127=ORIENTED_EDGE('',*,*,#46996,.F.);
#72128=ORIENTED_EDGE('',*,*,#51698,.F.);
#72129=ORIENTED_EDGE('',*,*,#49829,.F.);
#72130=ORIENTED_EDGE('',*,*,#51697,.T.);
#72131=ORIENTED_EDGE('',*,*,#49836,.F.);
#72132=ORIENTED_EDGE('',*,*,#51699,.F.);
#72133=ORIENTED_EDGE('',*,*,#47000,.F.);
#72134=ORIENTED_EDGE('',*,*,#51698,.T.);
#72135=ORIENTED_EDGE('',*,*,#46206,.F.);
#72136=ORIENTED_EDGE('',*,*,#51700,.F.);
#72137=ORIENTED_EDGE('',*,*,#49830,.F.);
#72138=ORIENTED_EDGE('',*,*,#51699,.T.);
#72139=ORIENTED_EDGE('',*,*,#49835,.F.);
#72140=ORIENTED_EDGE('',*,*,#51701,.F.);
#72141=ORIENTED_EDGE('',*,*,#46975,.T.);
#72142=ORIENTED_EDGE('',*,*,#46979,.F.);
#72143=ORIENTED_EDGE('',*,*,#51700,.T.);
#72144=ORIENTED_EDGE('',*,*,#46205,.F.);
#72145=ORIENTED_EDGE('',*,*,#51702,.F.);
#72146=ORIENTED_EDGE('',*,*,#50337,.F.);
#72147=ORIENTED_EDGE('',*,*,#51701,.T.);
#72148=ORIENTED_EDGE('',*,*,#49834,.F.);
#72149=ORIENTED_EDGE('',*,*,#51703,.F.);
#72150=ORIENTED_EDGE('',*,*,#46976,.F.);
#72151=ORIENTED_EDGE('',*,*,#51702,.T.);
#72152=ORIENTED_EDGE('',*,*,#46204,.F.);
#72153=ORIENTED_EDGE('',*,*,#51704,.F.);
#72154=ORIENTED_EDGE('',*,*,#49814,.F.);
#72155=ORIENTED_EDGE('',*,*,#51703,.T.);
#72156=ORIENTED_EDGE('',*,*,#49833,.F.);
#72157=ORIENTED_EDGE('',*,*,#51705,.F.);
#72158=ORIENTED_EDGE('',*,*,#46994,.F.);
#72159=ORIENTED_EDGE('',*,*,#51704,.T.);
#72160=ORIENTED_EDGE('',*,*,#46203,.F.);
#72161=ORIENTED_EDGE('',*,*,#51706,.F.);
#72162=ORIENTED_EDGE('',*,*,#50339,.F.);
#72163=ORIENTED_EDGE('',*,*,#51705,.T.);
#72164=ORIENTED_EDGE('',*,*,#49832,.F.);
#72165=ORIENTED_EDGE('',*,*,#51707,.F.);
#72166=ORIENTED_EDGE('',*,*,#46527,.F.);
#72167=ORIENTED_EDGE('',*,*,#51706,.T.);
#72168=ORIENTED_EDGE('',*,*,#46202,.F.);
#72169=ORIENTED_EDGE('',*,*,#51708,.F.);
#72170=ORIENTED_EDGE('',*,*,#49820,.F.);
#72171=ORIENTED_EDGE('',*,*,#51707,.T.);
#72172=ORIENTED_EDGE('',*,*,#50338,.F.);
#72173=ORIENTED_EDGE('',*,*,#51709,.F.);
#72174=ORIENTED_EDGE('',*,*,#46528,.F.);
#72175=ORIENTED_EDGE('',*,*,#51708,.T.);
#72176=ORIENTED_EDGE('',*,*,#47025,.F.);
#72177=ORIENTED_EDGE('',*,*,#51710,.F.);
#72178=ORIENTED_EDGE('',*,*,#49821,.F.);
#72179=ORIENTED_EDGE('',*,*,#51709,.T.);
#72180=ORIENTED_EDGE('',*,*,#49816,.F.);
#72181=ORIENTED_EDGE('',*,*,#51711,.F.);
#72182=ORIENTED_EDGE('',*,*,#46529,.F.);
#72183=ORIENTED_EDGE('',*,*,#47020,.F.);
#72184=ORIENTED_EDGE('',*,*,#47016,.T.);
#72185=ORIENTED_EDGE('',*,*,#51712,.F.);
#72186=ORIENTED_EDGE('',*,*,#49822,.F.);
#72187=ORIENTED_EDGE('',*,*,#51710,.T.);
#72188=ORIENTED_EDGE('',*,*,#51711,.T.);
#72189=ORIENTED_EDGE('',*,*,#50340,.F.);
#72190=ORIENTED_EDGE('',*,*,#51713,.F.);
#72191=ORIENTED_EDGE('',*,*,#46530,.F.);
#72192=ORIENTED_EDGE('',*,*,#51712,.T.);
#72193=ORIENTED_EDGE('',*,*,#47015,.F.);
#72194=ORIENTED_EDGE('',*,*,#51714,.F.);
#72195=ORIENTED_EDGE('',*,*,#49823,.F.);
#72196=ORIENTED_EDGE('',*,*,#51713,.T.);
#72197=ORIENTED_EDGE('',*,*,#49818,.F.);
#72198=ORIENTED_EDGE('',*,*,#51715,.F.);
#72199=ORIENTED_EDGE('',*,*,#46531,.F.);
#72200=ORIENTED_EDGE('',*,*,#51714,.T.);
#72201=ORIENTED_EDGE('',*,*,#47027,.F.);
#72202=ORIENTED_EDGE('',*,*,#51716,.F.);
#72203=ORIENTED_EDGE('',*,*,#49824,.F.);
#72204=ORIENTED_EDGE('',*,*,#51715,.T.);
#72205=ORIENTED_EDGE('',*,*,#49817,.F.);
#72206=ORIENTED_EDGE('',*,*,#51717,.F.);
#72207=ORIENTED_EDGE('',*,*,#47023,.F.);
#72208=ORIENTED_EDGE('',*,*,#51716,.T.);
#72209=ORIENTED_EDGE('',*,*,#47011,.F.);
#72210=ORIENTED_EDGE('',*,*,#51718,.F.);
#72211=ORIENTED_EDGE('',*,*,#49825,.F.);
#72212=ORIENTED_EDGE('',*,*,#51717,.T.);
#72213=ORIENTED_EDGE('',*,*,#49828,.F.);
#72214=ORIENTED_EDGE('',*,*,#51719,.F.);
#72215=ORIENTED_EDGE('',*,*,#47002,.F.);
#72216=ORIENTED_EDGE('',*,*,#51718,.T.);
#72217=ORIENTED_EDGE('',*,*,#47029,.F.);
#72218=ORIENTED_EDGE('',*,*,#51720,.F.);
#72219=ORIENTED_EDGE('',*,*,#49826,.F.);
#72220=ORIENTED_EDGE('',*,*,#51719,.T.);
#72221=ORIENTED_EDGE('',*,*,#49827,.F.);
#72222=ORIENTED_EDGE('',*,*,#51720,.T.);
#72223=ORIENTED_EDGE('',*,*,#47007,.F.);
#72224=ORIENTED_EDGE('',*,*,#47003,.T.);
#72225=ORIENTED_EDGE('',*,*,#51721,.F.);
#72226=ORIENTED_EDGE('',*,*,#49867,.F.);
#72227=ORIENTED_EDGE('',*,*,#51722,.F.);
#72228=ORIENTED_EDGE('',*,*,#46959,.F.);
#72229=ORIENTED_EDGE('',*,*,#51722,.T.);
#72230=ORIENTED_EDGE('',*,*,#49866,.F.);
#72231=ORIENTED_EDGE('',*,*,#51723,.F.);
#72232=ORIENTED_EDGE('',*,*,#46968,.F.);
#72233=ORIENTED_EDGE('',*,*,#46958,.T.);
#72234=ORIENTED_EDGE('',*,*,#46962,.F.);
#72235=ORIENTED_EDGE('',*,*,#51724,.F.);
#72236=ORIENTED_EDGE('',*,*,#49868,.F.);
#72237=ORIENTED_EDGE('',*,*,#51721,.T.);
#72238=ORIENTED_EDGE('',*,*,#51723,.T.);
#72239=ORIENTED_EDGE('',*,*,#49865,.F.);
#72240=ORIENTED_EDGE('',*,*,#51725,.F.);
#72241=ORIENTED_EDGE('',*,*,#46953,.F.);
#72242=ORIENTED_EDGE('',*,*,#51724,.T.);
#72243=ORIENTED_EDGE('',*,*,#46966,.F.);
#72244=ORIENTED_EDGE('',*,*,#51726,.F.);
#72245=ORIENTED_EDGE('',*,*,#49857,.F.);
#72246=ORIENTED_EDGE('',*,*,#51725,.T.);
#72247=ORIENTED_EDGE('',*,*,#49864,.F.);
#72248=ORIENTED_EDGE('',*,*,#51727,.F.);
#72249=ORIENTED_EDGE('',*,*,#46970,.F.);
#72250=ORIENTED_EDGE('',*,*,#51726,.T.);
#72251=ORIENTED_EDGE('',*,*,#46212,.F.);
#72252=ORIENTED_EDGE('',*,*,#51728,.F.);
#72253=ORIENTED_EDGE('',*,*,#49858,.F.);
#72254=ORIENTED_EDGE('',*,*,#51727,.T.);
#72255=ORIENTED_EDGE('',*,*,#49863,.F.);
#72256=ORIENTED_EDGE('',*,*,#51729,.F.);
#72257=ORIENTED_EDGE('',*,*,#46945,.T.);
#72258=ORIENTED_EDGE('',*,*,#46949,.F.);
#72259=ORIENTED_EDGE('',*,*,#51728,.T.);
#72260=ORIENTED_EDGE('',*,*,#46211,.F.);
#72261=ORIENTED_EDGE('',*,*,#51730,.F.);
#72262=ORIENTED_EDGE('',*,*,#50341,.F.);
#72263=ORIENTED_EDGE('',*,*,#51729,.T.);
#72264=ORIENTED_EDGE('',*,*,#49862,.F.);
#72265=ORIENTED_EDGE('',*,*,#51731,.F.);
#72266=ORIENTED_EDGE('',*,*,#46946,.F.);
#72267=ORIENTED_EDGE('',*,*,#51730,.T.);
#72268=ORIENTED_EDGE('',*,*,#46210,.F.);
#72269=ORIENTED_EDGE('',*,*,#51732,.F.);
#72270=ORIENTED_EDGE('',*,*,#49842,.F.);
#72271=ORIENTED_EDGE('',*,*,#51731,.T.);
#72272=ORIENTED_EDGE('',*,*,#49861,.F.);
#72273=ORIENTED_EDGE('',*,*,#51733,.F.);
#72274=ORIENTED_EDGE('',*,*,#46964,.F.);
#72275=ORIENTED_EDGE('',*,*,#51732,.T.);
#72276=ORIENTED_EDGE('',*,*,#46209,.F.);
#72277=ORIENTED_EDGE('',*,*,#51734,.F.);
#72278=ORIENTED_EDGE('',*,*,#50343,.F.);
#72279=ORIENTED_EDGE('',*,*,#51733,.T.);
#72280=ORIENTED_EDGE('',*,*,#49860,.F.);
#72281=ORIENTED_EDGE('',*,*,#51735,.F.);
#72282=ORIENTED_EDGE('',*,*,#46521,.F.);
#72283=ORIENTED_EDGE('',*,*,#51734,.T.);
#72284=ORIENTED_EDGE('',*,*,#46208,.F.);
#72285=ORIENTED_EDGE('',*,*,#51736,.F.);
#72286=ORIENTED_EDGE('',*,*,#49848,.F.);
#72287=ORIENTED_EDGE('',*,*,#51735,.T.);
#72288=ORIENTED_EDGE('',*,*,#50342,.F.);
#72289=ORIENTED_EDGE('',*,*,#51737,.F.);
#72290=ORIENTED_EDGE('',*,*,#46522,.F.);
#72291=ORIENTED_EDGE('',*,*,#51736,.T.);
#72292=ORIENTED_EDGE('',*,*,#46995,.F.);
#72293=ORIENTED_EDGE('',*,*,#51738,.F.);
#72294=ORIENTED_EDGE('',*,*,#49849,.F.);
#72295=ORIENTED_EDGE('',*,*,#51737,.T.);
#72296=ORIENTED_EDGE('',*,*,#49844,.F.);
#72297=ORIENTED_EDGE('',*,*,#51739,.F.);
#72298=ORIENTED_EDGE('',*,*,#46523,.F.);
#72299=ORIENTED_EDGE('',*,*,#46990,.F.);
#72300=ORIENTED_EDGE('',*,*,#46986,.T.);
#72301=ORIENTED_EDGE('',*,*,#51740,.F.);
#72302=ORIENTED_EDGE('',*,*,#49850,.F.);
#72303=ORIENTED_EDGE('',*,*,#51738,.T.);
#72304=ORIENTED_EDGE('',*,*,#51739,.T.);
#72305=ORIENTED_EDGE('',*,*,#50344,.F.);
#72306=ORIENTED_EDGE('',*,*,#51741,.F.);
#72307=ORIENTED_EDGE('',*,*,#46524,.F.);
#72308=ORIENTED_EDGE('',*,*,#51740,.T.);
#72309=ORIENTED_EDGE('',*,*,#46985,.F.);
#72310=ORIENTED_EDGE('',*,*,#51742,.F.);
#72311=ORIENTED_EDGE('',*,*,#49851,.F.);
#72312=ORIENTED_EDGE('',*,*,#51741,.T.);
#72313=ORIENTED_EDGE('',*,*,#49846,.F.);
#72314=ORIENTED_EDGE('',*,*,#51743,.F.);
#72315=ORIENTED_EDGE('',*,*,#46525,.F.);
#72316=ORIENTED_EDGE('',*,*,#51742,.T.);
#72317=ORIENTED_EDGE('',*,*,#46997,.F.);
#72318=ORIENTED_EDGE('',*,*,#51744,.F.);
#72319=ORIENTED_EDGE('',*,*,#49852,.F.);
#72320=ORIENTED_EDGE('',*,*,#51743,.T.);
#72321=ORIENTED_EDGE('',*,*,#49845,.F.);
#72322=ORIENTED_EDGE('',*,*,#51745,.F.);
#72323=ORIENTED_EDGE('',*,*,#46993,.F.);
#72324=ORIENTED_EDGE('',*,*,#51744,.T.);
#72325=ORIENTED_EDGE('',*,*,#46981,.F.);
#72326=ORIENTED_EDGE('',*,*,#51746,.F.);
#72327=ORIENTED_EDGE('',*,*,#49853,.F.);
#72328=ORIENTED_EDGE('',*,*,#51745,.T.);
#72329=ORIENTED_EDGE('',*,*,#49856,.F.);
#72330=ORIENTED_EDGE('',*,*,#51747,.F.);
#72331=ORIENTED_EDGE('',*,*,#46972,.F.);
#72332=ORIENTED_EDGE('',*,*,#51746,.T.);
#72333=ORIENTED_EDGE('',*,*,#46999,.F.);
#72334=ORIENTED_EDGE('',*,*,#51748,.F.);
#72335=ORIENTED_EDGE('',*,*,#49854,.F.);
#72336=ORIENTED_EDGE('',*,*,#51747,.T.);
#72337=ORIENTED_EDGE('',*,*,#49855,.F.);
#72338=ORIENTED_EDGE('',*,*,#51748,.T.);
#72339=ORIENTED_EDGE('',*,*,#46977,.F.);
#72340=ORIENTED_EDGE('',*,*,#46973,.T.);
#72341=ORIENTED_EDGE('',*,*,#51749,.F.);
#72342=ORIENTED_EDGE('',*,*,#49895,.F.);
#72343=ORIENTED_EDGE('',*,*,#51750,.F.);
#72344=ORIENTED_EDGE('',*,*,#46929,.F.);
#72345=ORIENTED_EDGE('',*,*,#51750,.T.);
#72346=ORIENTED_EDGE('',*,*,#49894,.F.);
#72347=ORIENTED_EDGE('',*,*,#51751,.F.);
#72348=ORIENTED_EDGE('',*,*,#46938,.F.);
#72349=ORIENTED_EDGE('',*,*,#46928,.T.);
#72350=ORIENTED_EDGE('',*,*,#46932,.F.);
#72351=ORIENTED_EDGE('',*,*,#51752,.F.);
#72352=ORIENTED_EDGE('',*,*,#49896,.F.);
#72353=ORIENTED_EDGE('',*,*,#51749,.T.);
#72354=ORIENTED_EDGE('',*,*,#51751,.T.);
#72355=ORIENTED_EDGE('',*,*,#49893,.F.);
#72356=ORIENTED_EDGE('',*,*,#51753,.F.);
#72357=ORIENTED_EDGE('',*,*,#46923,.F.);
#72358=ORIENTED_EDGE('',*,*,#51752,.T.);
#72359=ORIENTED_EDGE('',*,*,#46936,.F.);
#72360=ORIENTED_EDGE('',*,*,#51754,.F.);
#72361=ORIENTED_EDGE('',*,*,#49885,.F.);
#72362=ORIENTED_EDGE('',*,*,#51753,.T.);
#72363=ORIENTED_EDGE('',*,*,#49892,.F.);
#72364=ORIENTED_EDGE('',*,*,#51755,.F.);
#72365=ORIENTED_EDGE('',*,*,#46940,.F.);
#72366=ORIENTED_EDGE('',*,*,#51754,.T.);
#72367=ORIENTED_EDGE('',*,*,#46218,.F.);
#72368=ORIENTED_EDGE('',*,*,#51756,.F.);
#72369=ORIENTED_EDGE('',*,*,#49886,.F.);
#72370=ORIENTED_EDGE('',*,*,#51755,.T.);
#72371=ORIENTED_EDGE('',*,*,#49891,.F.);
#72372=ORIENTED_EDGE('',*,*,#51757,.F.);
#72373=ORIENTED_EDGE('',*,*,#46915,.T.);
#72374=ORIENTED_EDGE('',*,*,#46919,.F.);
#72375=ORIENTED_EDGE('',*,*,#51756,.T.);
#72376=ORIENTED_EDGE('',*,*,#46217,.F.);
#72377=ORIENTED_EDGE('',*,*,#51758,.F.);
#72378=ORIENTED_EDGE('',*,*,#50345,.F.);
#72379=ORIENTED_EDGE('',*,*,#51757,.T.);
#72380=ORIENTED_EDGE('',*,*,#49890,.F.);
#72381=ORIENTED_EDGE('',*,*,#51759,.F.);
#72382=ORIENTED_EDGE('',*,*,#46916,.F.);
#72383=ORIENTED_EDGE('',*,*,#51758,.T.);
#72384=ORIENTED_EDGE('',*,*,#46216,.F.);
#72385=ORIENTED_EDGE('',*,*,#51760,.F.);
#72386=ORIENTED_EDGE('',*,*,#49870,.F.);
#72387=ORIENTED_EDGE('',*,*,#51759,.T.);
#72388=ORIENTED_EDGE('',*,*,#49889,.F.);
#72389=ORIENTED_EDGE('',*,*,#51761,.F.);
#72390=ORIENTED_EDGE('',*,*,#46934,.F.);
#72391=ORIENTED_EDGE('',*,*,#51760,.T.);
#72392=ORIENTED_EDGE('',*,*,#46215,.F.);
#72393=ORIENTED_EDGE('',*,*,#51762,.F.);
#72394=ORIENTED_EDGE('',*,*,#50347,.F.);
#72395=ORIENTED_EDGE('',*,*,#51761,.T.);
#72396=ORIENTED_EDGE('',*,*,#49888,.F.);
#72397=ORIENTED_EDGE('',*,*,#51763,.F.);
#72398=ORIENTED_EDGE('',*,*,#46515,.F.);
#72399=ORIENTED_EDGE('',*,*,#51762,.T.);
#72400=ORIENTED_EDGE('',*,*,#46214,.F.);
#72401=ORIENTED_EDGE('',*,*,#51764,.F.);
#72402=ORIENTED_EDGE('',*,*,#49876,.F.);
#72403=ORIENTED_EDGE('',*,*,#51763,.T.);
#72404=ORIENTED_EDGE('',*,*,#50346,.F.);
#72405=ORIENTED_EDGE('',*,*,#51765,.F.);
#72406=ORIENTED_EDGE('',*,*,#46516,.F.);
#72407=ORIENTED_EDGE('',*,*,#51764,.T.);
#72408=ORIENTED_EDGE('',*,*,#46965,.F.);
#72409=ORIENTED_EDGE('',*,*,#51766,.F.);
#72410=ORIENTED_EDGE('',*,*,#49877,.F.);
#72411=ORIENTED_EDGE('',*,*,#51765,.T.);
#72412=ORIENTED_EDGE('',*,*,#49872,.F.);
#72413=ORIENTED_EDGE('',*,*,#51767,.F.);
#72414=ORIENTED_EDGE('',*,*,#46517,.F.);
#72415=ORIENTED_EDGE('',*,*,#46960,.F.);
#72416=ORIENTED_EDGE('',*,*,#46956,.T.);
#72417=ORIENTED_EDGE('',*,*,#51768,.F.);
#72418=ORIENTED_EDGE('',*,*,#49878,.F.);
#72419=ORIENTED_EDGE('',*,*,#51766,.T.);
#72420=ORIENTED_EDGE('',*,*,#51767,.T.);
#72421=ORIENTED_EDGE('',*,*,#50348,.F.);
#72422=ORIENTED_EDGE('',*,*,#51769,.F.);
#72423=ORIENTED_EDGE('',*,*,#46518,.F.);
#72424=ORIENTED_EDGE('',*,*,#51768,.T.);
#72425=ORIENTED_EDGE('',*,*,#46955,.F.);
#72426=ORIENTED_EDGE('',*,*,#51770,.F.);
#72427=ORIENTED_EDGE('',*,*,#49879,.F.);
#72428=ORIENTED_EDGE('',*,*,#51769,.T.);
#72429=ORIENTED_EDGE('',*,*,#49874,.F.);
#72430=ORIENTED_EDGE('',*,*,#51771,.F.);
#72431=ORIENTED_EDGE('',*,*,#46519,.F.);
#72432=ORIENTED_EDGE('',*,*,#51770,.T.);
#72433=ORIENTED_EDGE('',*,*,#46967,.F.);
#72434=ORIENTED_EDGE('',*,*,#51772,.F.);
#72435=ORIENTED_EDGE('',*,*,#49880,.F.);
#72436=ORIENTED_EDGE('',*,*,#51771,.T.);
#72437=ORIENTED_EDGE('',*,*,#49873,.F.);
#72438=ORIENTED_EDGE('',*,*,#51773,.F.);
#72439=ORIENTED_EDGE('',*,*,#46963,.F.);
#72440=ORIENTED_EDGE('',*,*,#51772,.T.);
#72441=ORIENTED_EDGE('',*,*,#46951,.F.);
#72442=ORIENTED_EDGE('',*,*,#51774,.F.);
#72443=ORIENTED_EDGE('',*,*,#49881,.F.);
#72444=ORIENTED_EDGE('',*,*,#51773,.T.);
#72445=ORIENTED_EDGE('',*,*,#49884,.F.);
#72446=ORIENTED_EDGE('',*,*,#51775,.F.);
#72447=ORIENTED_EDGE('',*,*,#46942,.F.);
#72448=ORIENTED_EDGE('',*,*,#51774,.T.);
#72449=ORIENTED_EDGE('',*,*,#46969,.F.);
#72450=ORIENTED_EDGE('',*,*,#51776,.F.);
#72451=ORIENTED_EDGE('',*,*,#49882,.F.);
#72452=ORIENTED_EDGE('',*,*,#51775,.T.);
#72453=ORIENTED_EDGE('',*,*,#49883,.F.);
#72454=ORIENTED_EDGE('',*,*,#51776,.T.);
#72455=ORIENTED_EDGE('',*,*,#46947,.F.);
#72456=ORIENTED_EDGE('',*,*,#46943,.T.);
#72457=ORIENTED_EDGE('',*,*,#51777,.F.);
#72458=ORIENTED_EDGE('',*,*,#49923,.F.);
#72459=ORIENTED_EDGE('',*,*,#51778,.F.);
#72460=ORIENTED_EDGE('',*,*,#46899,.F.);
#72461=ORIENTED_EDGE('',*,*,#51778,.T.);
#72462=ORIENTED_EDGE('',*,*,#49922,.F.);
#72463=ORIENTED_EDGE('',*,*,#51779,.F.);
#72464=ORIENTED_EDGE('',*,*,#46908,.F.);
#72465=ORIENTED_EDGE('',*,*,#46898,.T.);
#72466=ORIENTED_EDGE('',*,*,#46902,.F.);
#72467=ORIENTED_EDGE('',*,*,#51780,.F.);
#72468=ORIENTED_EDGE('',*,*,#49924,.F.);
#72469=ORIENTED_EDGE('',*,*,#51777,.T.);
#72470=ORIENTED_EDGE('',*,*,#51779,.T.);
#72471=ORIENTED_EDGE('',*,*,#49921,.F.);
#72472=ORIENTED_EDGE('',*,*,#51781,.F.);
#72473=ORIENTED_EDGE('',*,*,#46893,.F.);
#72474=ORIENTED_EDGE('',*,*,#51780,.T.);
#72475=ORIENTED_EDGE('',*,*,#46906,.F.);
#72476=ORIENTED_EDGE('',*,*,#51782,.F.);
#72477=ORIENTED_EDGE('',*,*,#49913,.F.);
#72478=ORIENTED_EDGE('',*,*,#51781,.T.);
#72479=ORIENTED_EDGE('',*,*,#49920,.F.);
#72480=ORIENTED_EDGE('',*,*,#51783,.F.);
#72481=ORIENTED_EDGE('',*,*,#46910,.F.);
#72482=ORIENTED_EDGE('',*,*,#51782,.T.);
#72483=ORIENTED_EDGE('',*,*,#46224,.F.);
#72484=ORIENTED_EDGE('',*,*,#51784,.F.);
#72485=ORIENTED_EDGE('',*,*,#49914,.F.);
#72486=ORIENTED_EDGE('',*,*,#51783,.T.);
#72487=ORIENTED_EDGE('',*,*,#49919,.F.);
#72488=ORIENTED_EDGE('',*,*,#51785,.F.);
#72489=ORIENTED_EDGE('',*,*,#46885,.T.);
#72490=ORIENTED_EDGE('',*,*,#46889,.F.);
#72491=ORIENTED_EDGE('',*,*,#51784,.T.);
#72492=ORIENTED_EDGE('',*,*,#46223,.F.);
#72493=ORIENTED_EDGE('',*,*,#51786,.F.);
#72494=ORIENTED_EDGE('',*,*,#50349,.F.);
#72495=ORIENTED_EDGE('',*,*,#51785,.T.);
#72496=ORIENTED_EDGE('',*,*,#49918,.F.);
#72497=ORIENTED_EDGE('',*,*,#51787,.F.);
#72498=ORIENTED_EDGE('',*,*,#46886,.F.);
#72499=ORIENTED_EDGE('',*,*,#51786,.T.);
#72500=ORIENTED_EDGE('',*,*,#46222,.F.);
#72501=ORIENTED_EDGE('',*,*,#51788,.F.);
#72502=ORIENTED_EDGE('',*,*,#49898,.F.);
#72503=ORIENTED_EDGE('',*,*,#51787,.T.);
#72504=ORIENTED_EDGE('',*,*,#49917,.F.);
#72505=ORIENTED_EDGE('',*,*,#51789,.F.);
#72506=ORIENTED_EDGE('',*,*,#46904,.F.);
#72507=ORIENTED_EDGE('',*,*,#51788,.T.);
#72508=ORIENTED_EDGE('',*,*,#46221,.F.);
#72509=ORIENTED_EDGE('',*,*,#51790,.F.);
#72510=ORIENTED_EDGE('',*,*,#50351,.F.);
#72511=ORIENTED_EDGE('',*,*,#51789,.T.);
#72512=ORIENTED_EDGE('',*,*,#49916,.F.);
#72513=ORIENTED_EDGE('',*,*,#51791,.F.);
#72514=ORIENTED_EDGE('',*,*,#46509,.F.);
#72515=ORIENTED_EDGE('',*,*,#51790,.T.);
#72516=ORIENTED_EDGE('',*,*,#46220,.F.);
#72517=ORIENTED_EDGE('',*,*,#51792,.F.);
#72518=ORIENTED_EDGE('',*,*,#49904,.F.);
#72519=ORIENTED_EDGE('',*,*,#51791,.T.);
#72520=ORIENTED_EDGE('',*,*,#50350,.F.);
#72521=ORIENTED_EDGE('',*,*,#51793,.F.);
#72522=ORIENTED_EDGE('',*,*,#46510,.F.);
#72523=ORIENTED_EDGE('',*,*,#51792,.T.);
#72524=ORIENTED_EDGE('',*,*,#46935,.F.);
#72525=ORIENTED_EDGE('',*,*,#51794,.F.);
#72526=ORIENTED_EDGE('',*,*,#49905,.F.);
#72527=ORIENTED_EDGE('',*,*,#51793,.T.);
#72528=ORIENTED_EDGE('',*,*,#49900,.F.);
#72529=ORIENTED_EDGE('',*,*,#51795,.F.);
#72530=ORIENTED_EDGE('',*,*,#46511,.F.);
#72531=ORIENTED_EDGE('',*,*,#46930,.F.);
#72532=ORIENTED_EDGE('',*,*,#46926,.T.);
#72533=ORIENTED_EDGE('',*,*,#51796,.F.);
#72534=ORIENTED_EDGE('',*,*,#49906,.F.);
#72535=ORIENTED_EDGE('',*,*,#51794,.T.);
#72536=ORIENTED_EDGE('',*,*,#51795,.T.);
#72537=ORIENTED_EDGE('',*,*,#50352,.F.);
#72538=ORIENTED_EDGE('',*,*,#51797,.F.);
#72539=ORIENTED_EDGE('',*,*,#46512,.F.);
#72540=ORIENTED_EDGE('',*,*,#51796,.T.);
#72541=ORIENTED_EDGE('',*,*,#46925,.F.);
#72542=ORIENTED_EDGE('',*,*,#51798,.F.);
#72543=ORIENTED_EDGE('',*,*,#49907,.F.);
#72544=ORIENTED_EDGE('',*,*,#51797,.T.);
#72545=ORIENTED_EDGE('',*,*,#49902,.F.);
#72546=ORIENTED_EDGE('',*,*,#51799,.F.);
#72547=ORIENTED_EDGE('',*,*,#46513,.F.);
#72548=ORIENTED_EDGE('',*,*,#51798,.T.);
#72549=ORIENTED_EDGE('',*,*,#46937,.F.);
#72550=ORIENTED_EDGE('',*,*,#51800,.F.);
#72551=ORIENTED_EDGE('',*,*,#49908,.F.);
#72552=ORIENTED_EDGE('',*,*,#51799,.T.);
#72553=ORIENTED_EDGE('',*,*,#49901,.F.);
#72554=ORIENTED_EDGE('',*,*,#51801,.F.);
#72555=ORIENTED_EDGE('',*,*,#46933,.F.);
#72556=ORIENTED_EDGE('',*,*,#51800,.T.);
#72557=ORIENTED_EDGE('',*,*,#46921,.F.);
#72558=ORIENTED_EDGE('',*,*,#51802,.F.);
#72559=ORIENTED_EDGE('',*,*,#49909,.F.);
#72560=ORIENTED_EDGE('',*,*,#51801,.T.);
#72561=ORIENTED_EDGE('',*,*,#49912,.F.);
#72562=ORIENTED_EDGE('',*,*,#51803,.F.);
#72563=ORIENTED_EDGE('',*,*,#46912,.F.);
#72564=ORIENTED_EDGE('',*,*,#51802,.T.);
#72565=ORIENTED_EDGE('',*,*,#46939,.F.);
#72566=ORIENTED_EDGE('',*,*,#51804,.F.);
#72567=ORIENTED_EDGE('',*,*,#49910,.F.);
#72568=ORIENTED_EDGE('',*,*,#51803,.T.);
#72569=ORIENTED_EDGE('',*,*,#49911,.F.);
#72570=ORIENTED_EDGE('',*,*,#51804,.T.);
#72571=ORIENTED_EDGE('',*,*,#46917,.F.);
#72572=ORIENTED_EDGE('',*,*,#46913,.T.);
#72573=ORIENTED_EDGE('',*,*,#51805,.F.);
#72574=ORIENTED_EDGE('',*,*,#49951,.F.);
#72575=ORIENTED_EDGE('',*,*,#51806,.F.);
#72576=ORIENTED_EDGE('',*,*,#46869,.F.);
#72577=ORIENTED_EDGE('',*,*,#51806,.T.);
#72578=ORIENTED_EDGE('',*,*,#49950,.F.);
#72579=ORIENTED_EDGE('',*,*,#51807,.F.);
#72580=ORIENTED_EDGE('',*,*,#46878,.F.);
#72581=ORIENTED_EDGE('',*,*,#46868,.T.);
#72582=ORIENTED_EDGE('',*,*,#46872,.F.);
#72583=ORIENTED_EDGE('',*,*,#51808,.F.);
#72584=ORIENTED_EDGE('',*,*,#49952,.F.);
#72585=ORIENTED_EDGE('',*,*,#51805,.T.);
#72586=ORIENTED_EDGE('',*,*,#51807,.T.);
#72587=ORIENTED_EDGE('',*,*,#49949,.F.);
#72588=ORIENTED_EDGE('',*,*,#51809,.F.);
#72589=ORIENTED_EDGE('',*,*,#46863,.F.);
#72590=ORIENTED_EDGE('',*,*,#51808,.T.);
#72591=ORIENTED_EDGE('',*,*,#46876,.F.);
#72592=ORIENTED_EDGE('',*,*,#51810,.F.);
#72593=ORIENTED_EDGE('',*,*,#49941,.F.);
#72594=ORIENTED_EDGE('',*,*,#51809,.T.);
#72595=ORIENTED_EDGE('',*,*,#49948,.F.);
#72596=ORIENTED_EDGE('',*,*,#51811,.F.);
#72597=ORIENTED_EDGE('',*,*,#46880,.F.);
#72598=ORIENTED_EDGE('',*,*,#51810,.T.);
#72599=ORIENTED_EDGE('',*,*,#46230,.F.);
#72600=ORIENTED_EDGE('',*,*,#51812,.F.);
#72601=ORIENTED_EDGE('',*,*,#49942,.F.);
#72602=ORIENTED_EDGE('',*,*,#51811,.T.);
#72603=ORIENTED_EDGE('',*,*,#49947,.F.);
#72604=ORIENTED_EDGE('',*,*,#51813,.F.);
#72605=ORIENTED_EDGE('',*,*,#46855,.T.);
#72606=ORIENTED_EDGE('',*,*,#46859,.F.);
#72607=ORIENTED_EDGE('',*,*,#51812,.T.);
#72608=ORIENTED_EDGE('',*,*,#46229,.F.);
#72609=ORIENTED_EDGE('',*,*,#51814,.F.);
#72610=ORIENTED_EDGE('',*,*,#50353,.F.);
#72611=ORIENTED_EDGE('',*,*,#51813,.T.);
#72612=ORIENTED_EDGE('',*,*,#49946,.F.);
#72613=ORIENTED_EDGE('',*,*,#51815,.F.);
#72614=ORIENTED_EDGE('',*,*,#46856,.F.);
#72615=ORIENTED_EDGE('',*,*,#51814,.T.);
#72616=ORIENTED_EDGE('',*,*,#46228,.F.);
#72617=ORIENTED_EDGE('',*,*,#51816,.F.);
#72618=ORIENTED_EDGE('',*,*,#49926,.F.);
#72619=ORIENTED_EDGE('',*,*,#51815,.T.);
#72620=ORIENTED_EDGE('',*,*,#49945,.F.);
#72621=ORIENTED_EDGE('',*,*,#51817,.F.);
#72622=ORIENTED_EDGE('',*,*,#46874,.F.);
#72623=ORIENTED_EDGE('',*,*,#51816,.T.);
#72624=ORIENTED_EDGE('',*,*,#46227,.F.);
#72625=ORIENTED_EDGE('',*,*,#51818,.F.);
#72626=ORIENTED_EDGE('',*,*,#50355,.F.);
#72627=ORIENTED_EDGE('',*,*,#51817,.T.);
#72628=ORIENTED_EDGE('',*,*,#49944,.F.);
#72629=ORIENTED_EDGE('',*,*,#51819,.F.);
#72630=ORIENTED_EDGE('',*,*,#46503,.F.);
#72631=ORIENTED_EDGE('',*,*,#51818,.T.);
#72632=ORIENTED_EDGE('',*,*,#46226,.F.);
#72633=ORIENTED_EDGE('',*,*,#51820,.F.);
#72634=ORIENTED_EDGE('',*,*,#49932,.F.);
#72635=ORIENTED_EDGE('',*,*,#51819,.T.);
#72636=ORIENTED_EDGE('',*,*,#50354,.F.);
#72637=ORIENTED_EDGE('',*,*,#51821,.F.);
#72638=ORIENTED_EDGE('',*,*,#46504,.F.);
#72639=ORIENTED_EDGE('',*,*,#51820,.T.);
#72640=ORIENTED_EDGE('',*,*,#46905,.F.);
#72641=ORIENTED_EDGE('',*,*,#51822,.F.);
#72642=ORIENTED_EDGE('',*,*,#49933,.F.);
#72643=ORIENTED_EDGE('',*,*,#51821,.T.);
#72644=ORIENTED_EDGE('',*,*,#49928,.F.);
#72645=ORIENTED_EDGE('',*,*,#51823,.F.);
#72646=ORIENTED_EDGE('',*,*,#46505,.F.);
#72647=ORIENTED_EDGE('',*,*,#46900,.F.);
#72648=ORIENTED_EDGE('',*,*,#46896,.T.);
#72649=ORIENTED_EDGE('',*,*,#51824,.F.);
#72650=ORIENTED_EDGE('',*,*,#49934,.F.);
#72651=ORIENTED_EDGE('',*,*,#51822,.T.);
#72652=ORIENTED_EDGE('',*,*,#51823,.T.);
#72653=ORIENTED_EDGE('',*,*,#50356,.F.);
#72654=ORIENTED_EDGE('',*,*,#51825,.F.);
#72655=ORIENTED_EDGE('',*,*,#46506,.F.);
#72656=ORIENTED_EDGE('',*,*,#51824,.T.);
#72657=ORIENTED_EDGE('',*,*,#46895,.F.);
#72658=ORIENTED_EDGE('',*,*,#51826,.F.);
#72659=ORIENTED_EDGE('',*,*,#49935,.F.);
#72660=ORIENTED_EDGE('',*,*,#51825,.T.);
#72661=ORIENTED_EDGE('',*,*,#49930,.F.);
#72662=ORIENTED_EDGE('',*,*,#51827,.F.);
#72663=ORIENTED_EDGE('',*,*,#46507,.F.);
#72664=ORIENTED_EDGE('',*,*,#51826,.T.);
#72665=ORIENTED_EDGE('',*,*,#46907,.F.);
#72666=ORIENTED_EDGE('',*,*,#51828,.F.);
#72667=ORIENTED_EDGE('',*,*,#49936,.F.);
#72668=ORIENTED_EDGE('',*,*,#51827,.T.);
#72669=ORIENTED_EDGE('',*,*,#49929,.F.);
#72670=ORIENTED_EDGE('',*,*,#51829,.F.);
#72671=ORIENTED_EDGE('',*,*,#46903,.F.);
#72672=ORIENTED_EDGE('',*,*,#51828,.T.);
#72673=ORIENTED_EDGE('',*,*,#46891,.F.);
#72674=ORIENTED_EDGE('',*,*,#51830,.F.);
#72675=ORIENTED_EDGE('',*,*,#49937,.F.);
#72676=ORIENTED_EDGE('',*,*,#51829,.T.);
#72677=ORIENTED_EDGE('',*,*,#49940,.F.);
#72678=ORIENTED_EDGE('',*,*,#51831,.F.);
#72679=ORIENTED_EDGE('',*,*,#46882,.F.);
#72680=ORIENTED_EDGE('',*,*,#51830,.T.);
#72681=ORIENTED_EDGE('',*,*,#46909,.F.);
#72682=ORIENTED_EDGE('',*,*,#51832,.F.);
#72683=ORIENTED_EDGE('',*,*,#49938,.F.);
#72684=ORIENTED_EDGE('',*,*,#51831,.T.);
#72685=ORIENTED_EDGE('',*,*,#49939,.F.);
#72686=ORIENTED_EDGE('',*,*,#51832,.T.);
#72687=ORIENTED_EDGE('',*,*,#46887,.F.);
#72688=ORIENTED_EDGE('',*,*,#46883,.T.);
#72689=ORIENTED_EDGE('',*,*,#51833,.F.);
#72690=ORIENTED_EDGE('',*,*,#49979,.F.);
#72691=ORIENTED_EDGE('',*,*,#51834,.F.);
#72692=ORIENTED_EDGE('',*,*,#46839,.F.);
#72693=ORIENTED_EDGE('',*,*,#51834,.T.);
#72694=ORIENTED_EDGE('',*,*,#49978,.F.);
#72695=ORIENTED_EDGE('',*,*,#51835,.F.);
#72696=ORIENTED_EDGE('',*,*,#46848,.F.);
#72697=ORIENTED_EDGE('',*,*,#46838,.T.);
#72698=ORIENTED_EDGE('',*,*,#46842,.F.);
#72699=ORIENTED_EDGE('',*,*,#51836,.F.);
#72700=ORIENTED_EDGE('',*,*,#49980,.F.);
#72701=ORIENTED_EDGE('',*,*,#51833,.T.);
#72702=ORIENTED_EDGE('',*,*,#51835,.T.);
#72703=ORIENTED_EDGE('',*,*,#49977,.F.);
#72704=ORIENTED_EDGE('',*,*,#51837,.F.);
#72705=ORIENTED_EDGE('',*,*,#46833,.F.);
#72706=ORIENTED_EDGE('',*,*,#51836,.T.);
#72707=ORIENTED_EDGE('',*,*,#46846,.F.);
#72708=ORIENTED_EDGE('',*,*,#51838,.F.);
#72709=ORIENTED_EDGE('',*,*,#49969,.F.);
#72710=ORIENTED_EDGE('',*,*,#51837,.T.);
#72711=ORIENTED_EDGE('',*,*,#49976,.F.);
#72712=ORIENTED_EDGE('',*,*,#51839,.F.);
#72713=ORIENTED_EDGE('',*,*,#46850,.F.);
#72714=ORIENTED_EDGE('',*,*,#51838,.T.);
#72715=ORIENTED_EDGE('',*,*,#46236,.F.);
#72716=ORIENTED_EDGE('',*,*,#51840,.F.);
#72717=ORIENTED_EDGE('',*,*,#49970,.F.);
#72718=ORIENTED_EDGE('',*,*,#51839,.T.);
#72719=ORIENTED_EDGE('',*,*,#49975,.F.);
#72720=ORIENTED_EDGE('',*,*,#51841,.F.);
#72721=ORIENTED_EDGE('',*,*,#46825,.T.);
#72722=ORIENTED_EDGE('',*,*,#46829,.F.);
#72723=ORIENTED_EDGE('',*,*,#51840,.T.);
#72724=ORIENTED_EDGE('',*,*,#46235,.F.);
#72725=ORIENTED_EDGE('',*,*,#51842,.F.);
#72726=ORIENTED_EDGE('',*,*,#50357,.F.);
#72727=ORIENTED_EDGE('',*,*,#51841,.T.);
#72728=ORIENTED_EDGE('',*,*,#49974,.F.);
#72729=ORIENTED_EDGE('',*,*,#51843,.F.);
#72730=ORIENTED_EDGE('',*,*,#46826,.F.);
#72731=ORIENTED_EDGE('',*,*,#51842,.T.);
#72732=ORIENTED_EDGE('',*,*,#46234,.F.);
#72733=ORIENTED_EDGE('',*,*,#51844,.F.);
#72734=ORIENTED_EDGE('',*,*,#49954,.F.);
#72735=ORIENTED_EDGE('',*,*,#51843,.T.);
#72736=ORIENTED_EDGE('',*,*,#49973,.F.);
#72737=ORIENTED_EDGE('',*,*,#51845,.F.);
#72738=ORIENTED_EDGE('',*,*,#46844,.F.);
#72739=ORIENTED_EDGE('',*,*,#51844,.T.);
#72740=ORIENTED_EDGE('',*,*,#46233,.F.);
#72741=ORIENTED_EDGE('',*,*,#51846,.F.);
#72742=ORIENTED_EDGE('',*,*,#50359,.F.);
#72743=ORIENTED_EDGE('',*,*,#51845,.T.);
#72744=ORIENTED_EDGE('',*,*,#49972,.F.);
#72745=ORIENTED_EDGE('',*,*,#51847,.F.);
#72746=ORIENTED_EDGE('',*,*,#46497,.F.);
#72747=ORIENTED_EDGE('',*,*,#51846,.T.);
#72748=ORIENTED_EDGE('',*,*,#46232,.F.);
#72749=ORIENTED_EDGE('',*,*,#51848,.F.);
#72750=ORIENTED_EDGE('',*,*,#49960,.F.);
#72751=ORIENTED_EDGE('',*,*,#51847,.T.);
#72752=ORIENTED_EDGE('',*,*,#50358,.F.);
#72753=ORIENTED_EDGE('',*,*,#51849,.F.);
#72754=ORIENTED_EDGE('',*,*,#46498,.F.);
#72755=ORIENTED_EDGE('',*,*,#51848,.T.);
#72756=ORIENTED_EDGE('',*,*,#46875,.F.);
#72757=ORIENTED_EDGE('',*,*,#51850,.F.);
#72758=ORIENTED_EDGE('',*,*,#49961,.F.);
#72759=ORIENTED_EDGE('',*,*,#51849,.T.);
#72760=ORIENTED_EDGE('',*,*,#49956,.F.);
#72761=ORIENTED_EDGE('',*,*,#51851,.F.);
#72762=ORIENTED_EDGE('',*,*,#46499,.F.);
#72763=ORIENTED_EDGE('',*,*,#46870,.F.);
#72764=ORIENTED_EDGE('',*,*,#46866,.T.);
#72765=ORIENTED_EDGE('',*,*,#51852,.F.);
#72766=ORIENTED_EDGE('',*,*,#49962,.F.);
#72767=ORIENTED_EDGE('',*,*,#51850,.T.);
#72768=ORIENTED_EDGE('',*,*,#51851,.T.);
#72769=ORIENTED_EDGE('',*,*,#50360,.F.);
#72770=ORIENTED_EDGE('',*,*,#51853,.F.);
#72771=ORIENTED_EDGE('',*,*,#46500,.F.);
#72772=ORIENTED_EDGE('',*,*,#51852,.T.);
#72773=ORIENTED_EDGE('',*,*,#46865,.F.);
#72774=ORIENTED_EDGE('',*,*,#51854,.F.);
#72775=ORIENTED_EDGE('',*,*,#49963,.F.);
#72776=ORIENTED_EDGE('',*,*,#51853,.T.);
#72777=ORIENTED_EDGE('',*,*,#49958,.F.);
#72778=ORIENTED_EDGE('',*,*,#51855,.F.);
#72779=ORIENTED_EDGE('',*,*,#46501,.F.);
#72780=ORIENTED_EDGE('',*,*,#51854,.T.);
#72781=ORIENTED_EDGE('',*,*,#46877,.F.);
#72782=ORIENTED_EDGE('',*,*,#51856,.F.);
#72783=ORIENTED_EDGE('',*,*,#49964,.F.);
#72784=ORIENTED_EDGE('',*,*,#51855,.T.);
#72785=ORIENTED_EDGE('',*,*,#49957,.F.);
#72786=ORIENTED_EDGE('',*,*,#51857,.F.);
#72787=ORIENTED_EDGE('',*,*,#46873,.F.);
#72788=ORIENTED_EDGE('',*,*,#51856,.T.);
#72789=ORIENTED_EDGE('',*,*,#46861,.F.);
#72790=ORIENTED_EDGE('',*,*,#51858,.F.);
#72791=ORIENTED_EDGE('',*,*,#49965,.F.);
#72792=ORIENTED_EDGE('',*,*,#51857,.T.);
#72793=ORIENTED_EDGE('',*,*,#49968,.F.);
#72794=ORIENTED_EDGE('',*,*,#51859,.F.);
#72795=ORIENTED_EDGE('',*,*,#46852,.F.);
#72796=ORIENTED_EDGE('',*,*,#51858,.T.);
#72797=ORIENTED_EDGE('',*,*,#46879,.F.);
#72798=ORIENTED_EDGE('',*,*,#51860,.F.);
#72799=ORIENTED_EDGE('',*,*,#49966,.F.);
#72800=ORIENTED_EDGE('',*,*,#51859,.T.);
#72801=ORIENTED_EDGE('',*,*,#49967,.F.);
#72802=ORIENTED_EDGE('',*,*,#51860,.T.);
#72803=ORIENTED_EDGE('',*,*,#46857,.F.);
#72804=ORIENTED_EDGE('',*,*,#46853,.T.);
#72805=ORIENTED_EDGE('',*,*,#51861,.F.);
#72806=ORIENTED_EDGE('',*,*,#50007,.F.);
#72807=ORIENTED_EDGE('',*,*,#51862,.F.);
#72808=ORIENTED_EDGE('',*,*,#46809,.F.);
#72809=ORIENTED_EDGE('',*,*,#51862,.T.);
#72810=ORIENTED_EDGE('',*,*,#50006,.F.);
#72811=ORIENTED_EDGE('',*,*,#51863,.F.);
#72812=ORIENTED_EDGE('',*,*,#46818,.F.);
#72813=ORIENTED_EDGE('',*,*,#46808,.T.);
#72814=ORIENTED_EDGE('',*,*,#46812,.F.);
#72815=ORIENTED_EDGE('',*,*,#51864,.F.);
#72816=ORIENTED_EDGE('',*,*,#50008,.F.);
#72817=ORIENTED_EDGE('',*,*,#51861,.T.);
#72818=ORIENTED_EDGE('',*,*,#51863,.T.);
#72819=ORIENTED_EDGE('',*,*,#50005,.F.);
#72820=ORIENTED_EDGE('',*,*,#51865,.F.);
#72821=ORIENTED_EDGE('',*,*,#46803,.F.);
#72822=ORIENTED_EDGE('',*,*,#51864,.T.);
#72823=ORIENTED_EDGE('',*,*,#46816,.F.);
#72824=ORIENTED_EDGE('',*,*,#51866,.F.);
#72825=ORIENTED_EDGE('',*,*,#49997,.F.);
#72826=ORIENTED_EDGE('',*,*,#51865,.T.);
#72827=ORIENTED_EDGE('',*,*,#50004,.F.);
#72828=ORIENTED_EDGE('',*,*,#51867,.F.);
#72829=ORIENTED_EDGE('',*,*,#46820,.F.);
#72830=ORIENTED_EDGE('',*,*,#51866,.T.);
#72831=ORIENTED_EDGE('',*,*,#46242,.F.);
#72832=ORIENTED_EDGE('',*,*,#51868,.F.);
#72833=ORIENTED_EDGE('',*,*,#49998,.F.);
#72834=ORIENTED_EDGE('',*,*,#51867,.T.);
#72835=ORIENTED_EDGE('',*,*,#50003,.F.);
#72836=ORIENTED_EDGE('',*,*,#51869,.F.);
#72837=ORIENTED_EDGE('',*,*,#46795,.T.);
#72838=ORIENTED_EDGE('',*,*,#46799,.F.);
#72839=ORIENTED_EDGE('',*,*,#51868,.T.);
#72840=ORIENTED_EDGE('',*,*,#46241,.F.);
#72841=ORIENTED_EDGE('',*,*,#51870,.F.);
#72842=ORIENTED_EDGE('',*,*,#50361,.F.);
#72843=ORIENTED_EDGE('',*,*,#51869,.T.);
#72844=ORIENTED_EDGE('',*,*,#50002,.F.);
#72845=ORIENTED_EDGE('',*,*,#51871,.F.);
#72846=ORIENTED_EDGE('',*,*,#46796,.F.);
#72847=ORIENTED_EDGE('',*,*,#51870,.T.);
#72848=ORIENTED_EDGE('',*,*,#46240,.F.);
#72849=ORIENTED_EDGE('',*,*,#51872,.F.);
#72850=ORIENTED_EDGE('',*,*,#49982,.F.);
#72851=ORIENTED_EDGE('',*,*,#51871,.T.);
#72852=ORIENTED_EDGE('',*,*,#50001,.F.);
#72853=ORIENTED_EDGE('',*,*,#51873,.F.);
#72854=ORIENTED_EDGE('',*,*,#46814,.F.);
#72855=ORIENTED_EDGE('',*,*,#51872,.T.);
#72856=ORIENTED_EDGE('',*,*,#46239,.F.);
#72857=ORIENTED_EDGE('',*,*,#51874,.F.);
#72858=ORIENTED_EDGE('',*,*,#50363,.F.);
#72859=ORIENTED_EDGE('',*,*,#51873,.T.);
#72860=ORIENTED_EDGE('',*,*,#50000,.F.);
#72861=ORIENTED_EDGE('',*,*,#51875,.F.);
#72862=ORIENTED_EDGE('',*,*,#46491,.F.);
#72863=ORIENTED_EDGE('',*,*,#51874,.T.);
#72864=ORIENTED_EDGE('',*,*,#46238,.F.);
#72865=ORIENTED_EDGE('',*,*,#51876,.F.);
#72866=ORIENTED_EDGE('',*,*,#49988,.F.);
#72867=ORIENTED_EDGE('',*,*,#51875,.T.);
#72868=ORIENTED_EDGE('',*,*,#50362,.F.);
#72869=ORIENTED_EDGE('',*,*,#51877,.F.);
#72870=ORIENTED_EDGE('',*,*,#46492,.F.);
#72871=ORIENTED_EDGE('',*,*,#51876,.T.);
#72872=ORIENTED_EDGE('',*,*,#46845,.F.);
#72873=ORIENTED_EDGE('',*,*,#51878,.F.);
#72874=ORIENTED_EDGE('',*,*,#49989,.F.);
#72875=ORIENTED_EDGE('',*,*,#51877,.T.);
#72876=ORIENTED_EDGE('',*,*,#49984,.F.);
#72877=ORIENTED_EDGE('',*,*,#51879,.F.);
#72878=ORIENTED_EDGE('',*,*,#46493,.F.);
#72879=ORIENTED_EDGE('',*,*,#46840,.F.);
#72880=ORIENTED_EDGE('',*,*,#46836,.T.);
#72881=ORIENTED_EDGE('',*,*,#51880,.F.);
#72882=ORIENTED_EDGE('',*,*,#49990,.F.);
#72883=ORIENTED_EDGE('',*,*,#51878,.T.);
#72884=ORIENTED_EDGE('',*,*,#51879,.T.);
#72885=ORIENTED_EDGE('',*,*,#50364,.F.);
#72886=ORIENTED_EDGE('',*,*,#51881,.F.);
#72887=ORIENTED_EDGE('',*,*,#46494,.F.);
#72888=ORIENTED_EDGE('',*,*,#51880,.T.);
#72889=ORIENTED_EDGE('',*,*,#46835,.F.);
#72890=ORIENTED_EDGE('',*,*,#51882,.F.);
#72891=ORIENTED_EDGE('',*,*,#49991,.F.);
#72892=ORIENTED_EDGE('',*,*,#51881,.T.);
#72893=ORIENTED_EDGE('',*,*,#49986,.F.);
#72894=ORIENTED_EDGE('',*,*,#51883,.F.);
#72895=ORIENTED_EDGE('',*,*,#46495,.F.);
#72896=ORIENTED_EDGE('',*,*,#51882,.T.);
#72897=ORIENTED_EDGE('',*,*,#46847,.F.);
#72898=ORIENTED_EDGE('',*,*,#51884,.F.);
#72899=ORIENTED_EDGE('',*,*,#49992,.F.);
#72900=ORIENTED_EDGE('',*,*,#51883,.T.);
#72901=ORIENTED_EDGE('',*,*,#49985,.F.);
#72902=ORIENTED_EDGE('',*,*,#51885,.F.);
#72903=ORIENTED_EDGE('',*,*,#46843,.F.);
#72904=ORIENTED_EDGE('',*,*,#51884,.T.);
#72905=ORIENTED_EDGE('',*,*,#46831,.F.);
#72906=ORIENTED_EDGE('',*,*,#51886,.F.);
#72907=ORIENTED_EDGE('',*,*,#49993,.F.);
#72908=ORIENTED_EDGE('',*,*,#51885,.T.);
#72909=ORIENTED_EDGE('',*,*,#49996,.F.);
#72910=ORIENTED_EDGE('',*,*,#51887,.F.);
#72911=ORIENTED_EDGE('',*,*,#46822,.F.);
#72912=ORIENTED_EDGE('',*,*,#51886,.T.);
#72913=ORIENTED_EDGE('',*,*,#46849,.F.);
#72914=ORIENTED_EDGE('',*,*,#51888,.F.);
#72915=ORIENTED_EDGE('',*,*,#49994,.F.);
#72916=ORIENTED_EDGE('',*,*,#51887,.T.);
#72917=ORIENTED_EDGE('',*,*,#49995,.F.);
#72918=ORIENTED_EDGE('',*,*,#51888,.T.);
#72919=ORIENTED_EDGE('',*,*,#46827,.F.);
#72920=ORIENTED_EDGE('',*,*,#46823,.T.);
#72921=ORIENTED_EDGE('',*,*,#51889,.F.);
#72922=ORIENTED_EDGE('',*,*,#50035,.F.);
#72923=ORIENTED_EDGE('',*,*,#51890,.F.);
#72924=ORIENTED_EDGE('',*,*,#46779,.F.);
#72925=ORIENTED_EDGE('',*,*,#51890,.T.);
#72926=ORIENTED_EDGE('',*,*,#50034,.F.);
#72927=ORIENTED_EDGE('',*,*,#51891,.F.);
#72928=ORIENTED_EDGE('',*,*,#46788,.F.);
#72929=ORIENTED_EDGE('',*,*,#46778,.T.);
#72930=ORIENTED_EDGE('',*,*,#46782,.F.);
#72931=ORIENTED_EDGE('',*,*,#51892,.F.);
#72932=ORIENTED_EDGE('',*,*,#50036,.F.);
#72933=ORIENTED_EDGE('',*,*,#51889,.T.);
#72934=ORIENTED_EDGE('',*,*,#51891,.T.);
#72935=ORIENTED_EDGE('',*,*,#50033,.F.);
#72936=ORIENTED_EDGE('',*,*,#51893,.F.);
#72937=ORIENTED_EDGE('',*,*,#46773,.F.);
#72938=ORIENTED_EDGE('',*,*,#51892,.T.);
#72939=ORIENTED_EDGE('',*,*,#46786,.F.);
#72940=ORIENTED_EDGE('',*,*,#51894,.F.);
#72941=ORIENTED_EDGE('',*,*,#50025,.F.);
#72942=ORIENTED_EDGE('',*,*,#51893,.T.);
#72943=ORIENTED_EDGE('',*,*,#50032,.F.);
#72944=ORIENTED_EDGE('',*,*,#51895,.F.);
#72945=ORIENTED_EDGE('',*,*,#46790,.F.);
#72946=ORIENTED_EDGE('',*,*,#51894,.T.);
#72947=ORIENTED_EDGE('',*,*,#46248,.F.);
#72948=ORIENTED_EDGE('',*,*,#51896,.F.);
#72949=ORIENTED_EDGE('',*,*,#50026,.F.);
#72950=ORIENTED_EDGE('',*,*,#51895,.T.);
#72951=ORIENTED_EDGE('',*,*,#50031,.F.);
#72952=ORIENTED_EDGE('',*,*,#51897,.F.);
#72953=ORIENTED_EDGE('',*,*,#46765,.T.);
#72954=ORIENTED_EDGE('',*,*,#46769,.F.);
#72955=ORIENTED_EDGE('',*,*,#51896,.T.);
#72956=ORIENTED_EDGE('',*,*,#46247,.F.);
#72957=ORIENTED_EDGE('',*,*,#51898,.F.);
#72958=ORIENTED_EDGE('',*,*,#50365,.F.);
#72959=ORIENTED_EDGE('',*,*,#51897,.T.);
#72960=ORIENTED_EDGE('',*,*,#50030,.F.);
#72961=ORIENTED_EDGE('',*,*,#51899,.F.);
#72962=ORIENTED_EDGE('',*,*,#46766,.F.);
#72963=ORIENTED_EDGE('',*,*,#51898,.T.);
#72964=ORIENTED_EDGE('',*,*,#46246,.F.);
#72965=ORIENTED_EDGE('',*,*,#51900,.F.);
#72966=ORIENTED_EDGE('',*,*,#50010,.F.);
#72967=ORIENTED_EDGE('',*,*,#51899,.T.);
#72968=ORIENTED_EDGE('',*,*,#50029,.F.);
#72969=ORIENTED_EDGE('',*,*,#51901,.F.);
#72970=ORIENTED_EDGE('',*,*,#46784,.F.);
#72971=ORIENTED_EDGE('',*,*,#51900,.T.);
#72972=ORIENTED_EDGE('',*,*,#46245,.F.);
#72973=ORIENTED_EDGE('',*,*,#51902,.F.);
#72974=ORIENTED_EDGE('',*,*,#50367,.F.);
#72975=ORIENTED_EDGE('',*,*,#51901,.T.);
#72976=ORIENTED_EDGE('',*,*,#50028,.F.);
#72977=ORIENTED_EDGE('',*,*,#51903,.F.);
#72978=ORIENTED_EDGE('',*,*,#46485,.F.);
#72979=ORIENTED_EDGE('',*,*,#51902,.T.);
#72980=ORIENTED_EDGE('',*,*,#46244,.F.);
#72981=ORIENTED_EDGE('',*,*,#51904,.F.);
#72982=ORIENTED_EDGE('',*,*,#50016,.F.);
#72983=ORIENTED_EDGE('',*,*,#51903,.T.);
#72984=ORIENTED_EDGE('',*,*,#50366,.F.);
#72985=ORIENTED_EDGE('',*,*,#51905,.F.);
#72986=ORIENTED_EDGE('',*,*,#46486,.F.);
#72987=ORIENTED_EDGE('',*,*,#51904,.T.);
#72988=ORIENTED_EDGE('',*,*,#46815,.F.);
#72989=ORIENTED_EDGE('',*,*,#51906,.F.);
#72990=ORIENTED_EDGE('',*,*,#50017,.F.);
#72991=ORIENTED_EDGE('',*,*,#51905,.T.);
#72992=ORIENTED_EDGE('',*,*,#50012,.F.);
#72993=ORIENTED_EDGE('',*,*,#51907,.F.);
#72994=ORIENTED_EDGE('',*,*,#46487,.F.);
#72995=ORIENTED_EDGE('',*,*,#46810,.F.);
#72996=ORIENTED_EDGE('',*,*,#46806,.T.);
#72997=ORIENTED_EDGE('',*,*,#51908,.F.);
#72998=ORIENTED_EDGE('',*,*,#50018,.F.);
#72999=ORIENTED_EDGE('',*,*,#51906,.T.);
#73000=ORIENTED_EDGE('',*,*,#51907,.T.);
#73001=ORIENTED_EDGE('',*,*,#50368,.F.);
#73002=ORIENTED_EDGE('',*,*,#51909,.F.);
#73003=ORIENTED_EDGE('',*,*,#46488,.F.);
#73004=ORIENTED_EDGE('',*,*,#51908,.T.);
#73005=ORIENTED_EDGE('',*,*,#46805,.F.);
#73006=ORIENTED_EDGE('',*,*,#51910,.F.);
#73007=ORIENTED_EDGE('',*,*,#50019,.F.);
#73008=ORIENTED_EDGE('',*,*,#51909,.T.);
#73009=ORIENTED_EDGE('',*,*,#50014,.F.);
#73010=ORIENTED_EDGE('',*,*,#51911,.F.);
#73011=ORIENTED_EDGE('',*,*,#46489,.F.);
#73012=ORIENTED_EDGE('',*,*,#51910,.T.);
#73013=ORIENTED_EDGE('',*,*,#46817,.F.);
#73014=ORIENTED_EDGE('',*,*,#51912,.F.);
#73015=ORIENTED_EDGE('',*,*,#50020,.F.);
#73016=ORIENTED_EDGE('',*,*,#51911,.T.);
#73017=ORIENTED_EDGE('',*,*,#50013,.F.);
#73018=ORIENTED_EDGE('',*,*,#51913,.F.);
#73019=ORIENTED_EDGE('',*,*,#46813,.F.);
#73020=ORIENTED_EDGE('',*,*,#51912,.T.);
#73021=ORIENTED_EDGE('',*,*,#46801,.F.);
#73022=ORIENTED_EDGE('',*,*,#51914,.F.);
#73023=ORIENTED_EDGE('',*,*,#50021,.F.);
#73024=ORIENTED_EDGE('',*,*,#51913,.T.);
#73025=ORIENTED_EDGE('',*,*,#50024,.F.);
#73026=ORIENTED_EDGE('',*,*,#51915,.F.);
#73027=ORIENTED_EDGE('',*,*,#46792,.F.);
#73028=ORIENTED_EDGE('',*,*,#51914,.T.);
#73029=ORIENTED_EDGE('',*,*,#46819,.F.);
#73030=ORIENTED_EDGE('',*,*,#51916,.F.);
#73031=ORIENTED_EDGE('',*,*,#50022,.F.);
#73032=ORIENTED_EDGE('',*,*,#51915,.T.);
#73033=ORIENTED_EDGE('',*,*,#50023,.F.);
#73034=ORIENTED_EDGE('',*,*,#51916,.T.);
#73035=ORIENTED_EDGE('',*,*,#46797,.F.);
#73036=ORIENTED_EDGE('',*,*,#46793,.T.);
#73037=ORIENTED_EDGE('',*,*,#51917,.F.);
#73038=ORIENTED_EDGE('',*,*,#50063,.F.);
#73039=ORIENTED_EDGE('',*,*,#51918,.F.);
#73040=ORIENTED_EDGE('',*,*,#46749,.F.);
#73041=ORIENTED_EDGE('',*,*,#51918,.T.);
#73042=ORIENTED_EDGE('',*,*,#50062,.F.);
#73043=ORIENTED_EDGE('',*,*,#51919,.F.);
#73044=ORIENTED_EDGE('',*,*,#46758,.F.);
#73045=ORIENTED_EDGE('',*,*,#46748,.T.);
#73046=ORIENTED_EDGE('',*,*,#46752,.F.);
#73047=ORIENTED_EDGE('',*,*,#51920,.F.);
#73048=ORIENTED_EDGE('',*,*,#50064,.F.);
#73049=ORIENTED_EDGE('',*,*,#51917,.T.);
#73050=ORIENTED_EDGE('',*,*,#51919,.T.);
#73051=ORIENTED_EDGE('',*,*,#50061,.F.);
#73052=ORIENTED_EDGE('',*,*,#51921,.F.);
#73053=ORIENTED_EDGE('',*,*,#46743,.F.);
#73054=ORIENTED_EDGE('',*,*,#51920,.T.);
#73055=ORIENTED_EDGE('',*,*,#46756,.F.);
#73056=ORIENTED_EDGE('',*,*,#51922,.F.);
#73057=ORIENTED_EDGE('',*,*,#50053,.F.);
#73058=ORIENTED_EDGE('',*,*,#51921,.T.);
#73059=ORIENTED_EDGE('',*,*,#50060,.F.);
#73060=ORIENTED_EDGE('',*,*,#51923,.F.);
#73061=ORIENTED_EDGE('',*,*,#46760,.F.);
#73062=ORIENTED_EDGE('',*,*,#51922,.T.);
#73063=ORIENTED_EDGE('',*,*,#46254,.F.);
#73064=ORIENTED_EDGE('',*,*,#51924,.F.);
#73065=ORIENTED_EDGE('',*,*,#50054,.F.);
#73066=ORIENTED_EDGE('',*,*,#51923,.T.);
#73067=ORIENTED_EDGE('',*,*,#50059,.F.);
#73068=ORIENTED_EDGE('',*,*,#51925,.F.);
#73069=ORIENTED_EDGE('',*,*,#46735,.T.);
#73070=ORIENTED_EDGE('',*,*,#46739,.F.);
#73071=ORIENTED_EDGE('',*,*,#51924,.T.);
#73072=ORIENTED_EDGE('',*,*,#46253,.F.);
#73073=ORIENTED_EDGE('',*,*,#51926,.F.);
#73074=ORIENTED_EDGE('',*,*,#50369,.F.);
#73075=ORIENTED_EDGE('',*,*,#51925,.T.);
#73076=ORIENTED_EDGE('',*,*,#50058,.F.);
#73077=ORIENTED_EDGE('',*,*,#51927,.F.);
#73078=ORIENTED_EDGE('',*,*,#46736,.F.);
#73079=ORIENTED_EDGE('',*,*,#51926,.T.);
#73080=ORIENTED_EDGE('',*,*,#46252,.F.);
#73081=ORIENTED_EDGE('',*,*,#51928,.F.);
#73082=ORIENTED_EDGE('',*,*,#50038,.F.);
#73083=ORIENTED_EDGE('',*,*,#51927,.T.);
#73084=ORIENTED_EDGE('',*,*,#50057,.F.);
#73085=ORIENTED_EDGE('',*,*,#51929,.F.);
#73086=ORIENTED_EDGE('',*,*,#46754,.F.);
#73087=ORIENTED_EDGE('',*,*,#51928,.T.);
#73088=ORIENTED_EDGE('',*,*,#46251,.F.);
#73089=ORIENTED_EDGE('',*,*,#51930,.F.);
#73090=ORIENTED_EDGE('',*,*,#50371,.F.);
#73091=ORIENTED_EDGE('',*,*,#51929,.T.);
#73092=ORIENTED_EDGE('',*,*,#50056,.F.);
#73093=ORIENTED_EDGE('',*,*,#51931,.F.);
#73094=ORIENTED_EDGE('',*,*,#46479,.F.);
#73095=ORIENTED_EDGE('',*,*,#51930,.T.);
#73096=ORIENTED_EDGE('',*,*,#46250,.F.);
#73097=ORIENTED_EDGE('',*,*,#51932,.F.);
#73098=ORIENTED_EDGE('',*,*,#50044,.F.);
#73099=ORIENTED_EDGE('',*,*,#51931,.T.);
#73100=ORIENTED_EDGE('',*,*,#50370,.F.);
#73101=ORIENTED_EDGE('',*,*,#51933,.F.);
#73102=ORIENTED_EDGE('',*,*,#46480,.F.);
#73103=ORIENTED_EDGE('',*,*,#51932,.T.);
#73104=ORIENTED_EDGE('',*,*,#46785,.F.);
#73105=ORIENTED_EDGE('',*,*,#51934,.F.);
#73106=ORIENTED_EDGE('',*,*,#50045,.F.);
#73107=ORIENTED_EDGE('',*,*,#51933,.T.);
#73108=ORIENTED_EDGE('',*,*,#50040,.F.);
#73109=ORIENTED_EDGE('',*,*,#51935,.F.);
#73110=ORIENTED_EDGE('',*,*,#46481,.F.);
#73111=ORIENTED_EDGE('',*,*,#46780,.F.);
#73112=ORIENTED_EDGE('',*,*,#46776,.T.);
#73113=ORIENTED_EDGE('',*,*,#51936,.F.);
#73114=ORIENTED_EDGE('',*,*,#50046,.F.);
#73115=ORIENTED_EDGE('',*,*,#51934,.T.);
#73116=ORIENTED_EDGE('',*,*,#51935,.T.);
#73117=ORIENTED_EDGE('',*,*,#50372,.F.);
#73118=ORIENTED_EDGE('',*,*,#51937,.F.);
#73119=ORIENTED_EDGE('',*,*,#46482,.F.);
#73120=ORIENTED_EDGE('',*,*,#51936,.T.);
#73121=ORIENTED_EDGE('',*,*,#46775,.F.);
#73122=ORIENTED_EDGE('',*,*,#51938,.F.);
#73123=ORIENTED_EDGE('',*,*,#50047,.F.);
#73124=ORIENTED_EDGE('',*,*,#51937,.T.);
#73125=ORIENTED_EDGE('',*,*,#50042,.F.);
#73126=ORIENTED_EDGE('',*,*,#51939,.F.);
#73127=ORIENTED_EDGE('',*,*,#46483,.F.);
#73128=ORIENTED_EDGE('',*,*,#51938,.T.);
#73129=ORIENTED_EDGE('',*,*,#46787,.F.);
#73130=ORIENTED_EDGE('',*,*,#51940,.F.);
#73131=ORIENTED_EDGE('',*,*,#50048,.F.);
#73132=ORIENTED_EDGE('',*,*,#51939,.T.);
#73133=ORIENTED_EDGE('',*,*,#50041,.F.);
#73134=ORIENTED_EDGE('',*,*,#51941,.F.);
#73135=ORIENTED_EDGE('',*,*,#46783,.F.);
#73136=ORIENTED_EDGE('',*,*,#51940,.T.);
#73137=ORIENTED_EDGE('',*,*,#46771,.F.);
#73138=ORIENTED_EDGE('',*,*,#51942,.F.);
#73139=ORIENTED_EDGE('',*,*,#50049,.F.);
#73140=ORIENTED_EDGE('',*,*,#51941,.T.);
#73141=ORIENTED_EDGE('',*,*,#50052,.F.);
#73142=ORIENTED_EDGE('',*,*,#51943,.F.);
#73143=ORIENTED_EDGE('',*,*,#46762,.F.);
#73144=ORIENTED_EDGE('',*,*,#51942,.T.);
#73145=ORIENTED_EDGE('',*,*,#46789,.F.);
#73146=ORIENTED_EDGE('',*,*,#51944,.F.);
#73147=ORIENTED_EDGE('',*,*,#50050,.F.);
#73148=ORIENTED_EDGE('',*,*,#51943,.T.);
#73149=ORIENTED_EDGE('',*,*,#50051,.F.);
#73150=ORIENTED_EDGE('',*,*,#51944,.T.);
#73151=ORIENTED_EDGE('',*,*,#46767,.F.);
#73152=ORIENTED_EDGE('',*,*,#46763,.T.);
#73153=ORIENTED_EDGE('',*,*,#51945,.F.);
#73154=ORIENTED_EDGE('',*,*,#50091,.F.);
#73155=ORIENTED_EDGE('',*,*,#51946,.F.);
#73156=ORIENTED_EDGE('',*,*,#46719,.F.);
#73157=ORIENTED_EDGE('',*,*,#51946,.T.);
#73158=ORIENTED_EDGE('',*,*,#50090,.F.);
#73159=ORIENTED_EDGE('',*,*,#51947,.F.);
#73160=ORIENTED_EDGE('',*,*,#46728,.F.);
#73161=ORIENTED_EDGE('',*,*,#46718,.T.);
#73162=ORIENTED_EDGE('',*,*,#46722,.F.);
#73163=ORIENTED_EDGE('',*,*,#51948,.F.);
#73164=ORIENTED_EDGE('',*,*,#50092,.F.);
#73165=ORIENTED_EDGE('',*,*,#51945,.T.);
#73166=ORIENTED_EDGE('',*,*,#51947,.T.);
#73167=ORIENTED_EDGE('',*,*,#50089,.F.);
#73168=ORIENTED_EDGE('',*,*,#51949,.F.);
#73169=ORIENTED_EDGE('',*,*,#46713,.F.);
#73170=ORIENTED_EDGE('',*,*,#51948,.T.);
#73171=ORIENTED_EDGE('',*,*,#46726,.F.);
#73172=ORIENTED_EDGE('',*,*,#51950,.F.);
#73173=ORIENTED_EDGE('',*,*,#50081,.F.);
#73174=ORIENTED_EDGE('',*,*,#51949,.T.);
#73175=ORIENTED_EDGE('',*,*,#50088,.F.);
#73176=ORIENTED_EDGE('',*,*,#51951,.F.);
#73177=ORIENTED_EDGE('',*,*,#46730,.F.);
#73178=ORIENTED_EDGE('',*,*,#51950,.T.);
#73179=ORIENTED_EDGE('',*,*,#46260,.F.);
#73180=ORIENTED_EDGE('',*,*,#51952,.F.);
#73181=ORIENTED_EDGE('',*,*,#50082,.F.);
#73182=ORIENTED_EDGE('',*,*,#51951,.T.);
#73183=ORIENTED_EDGE('',*,*,#50087,.F.);
#73184=ORIENTED_EDGE('',*,*,#51953,.F.);
#73185=ORIENTED_EDGE('',*,*,#46705,.T.);
#73186=ORIENTED_EDGE('',*,*,#46709,.F.);
#73187=ORIENTED_EDGE('',*,*,#51952,.T.);
#73188=ORIENTED_EDGE('',*,*,#46259,.F.);
#73189=ORIENTED_EDGE('',*,*,#51954,.F.);
#73190=ORIENTED_EDGE('',*,*,#50373,.F.);
#73191=ORIENTED_EDGE('',*,*,#51953,.T.);
#73192=ORIENTED_EDGE('',*,*,#50086,.F.);
#73193=ORIENTED_EDGE('',*,*,#51955,.F.);
#73194=ORIENTED_EDGE('',*,*,#46706,.F.);
#73195=ORIENTED_EDGE('',*,*,#51954,.T.);
#73196=ORIENTED_EDGE('',*,*,#46258,.F.);
#73197=ORIENTED_EDGE('',*,*,#51956,.F.);
#73198=ORIENTED_EDGE('',*,*,#50066,.F.);
#73199=ORIENTED_EDGE('',*,*,#51955,.T.);
#73200=ORIENTED_EDGE('',*,*,#50085,.F.);
#73201=ORIENTED_EDGE('',*,*,#51957,.F.);
#73202=ORIENTED_EDGE('',*,*,#46724,.F.);
#73203=ORIENTED_EDGE('',*,*,#51956,.T.);
#73204=ORIENTED_EDGE('',*,*,#46257,.F.);
#73205=ORIENTED_EDGE('',*,*,#51958,.F.);
#73206=ORIENTED_EDGE('',*,*,#50375,.F.);
#73207=ORIENTED_EDGE('',*,*,#51957,.T.);
#73208=ORIENTED_EDGE('',*,*,#50084,.F.);
#73209=ORIENTED_EDGE('',*,*,#51959,.F.);
#73210=ORIENTED_EDGE('',*,*,#46473,.F.);
#73211=ORIENTED_EDGE('',*,*,#51958,.T.);
#73212=ORIENTED_EDGE('',*,*,#46256,.F.);
#73213=ORIENTED_EDGE('',*,*,#51960,.F.);
#73214=ORIENTED_EDGE('',*,*,#50072,.F.);
#73215=ORIENTED_EDGE('',*,*,#51959,.T.);
#73216=ORIENTED_EDGE('',*,*,#50374,.F.);
#73217=ORIENTED_EDGE('',*,*,#51961,.F.);
#73218=ORIENTED_EDGE('',*,*,#46474,.F.);
#73219=ORIENTED_EDGE('',*,*,#51960,.T.);
#73220=ORIENTED_EDGE('',*,*,#46755,.F.);
#73221=ORIENTED_EDGE('',*,*,#51962,.F.);
#73222=ORIENTED_EDGE('',*,*,#50073,.F.);
#73223=ORIENTED_EDGE('',*,*,#51961,.T.);
#73224=ORIENTED_EDGE('',*,*,#50068,.F.);
#73225=ORIENTED_EDGE('',*,*,#51963,.F.);
#73226=ORIENTED_EDGE('',*,*,#46475,.F.);
#73227=ORIENTED_EDGE('',*,*,#46750,.F.);
#73228=ORIENTED_EDGE('',*,*,#46746,.T.);
#73229=ORIENTED_EDGE('',*,*,#51964,.F.);
#73230=ORIENTED_EDGE('',*,*,#50074,.F.);
#73231=ORIENTED_EDGE('',*,*,#51962,.T.);
#73232=ORIENTED_EDGE('',*,*,#51963,.T.);
#73233=ORIENTED_EDGE('',*,*,#50376,.F.);
#73234=ORIENTED_EDGE('',*,*,#51965,.F.);
#73235=ORIENTED_EDGE('',*,*,#46476,.F.);
#73236=ORIENTED_EDGE('',*,*,#51964,.T.);
#73237=ORIENTED_EDGE('',*,*,#46745,.F.);
#73238=ORIENTED_EDGE('',*,*,#51966,.F.);
#73239=ORIENTED_EDGE('',*,*,#50075,.F.);
#73240=ORIENTED_EDGE('',*,*,#51965,.T.);
#73241=ORIENTED_EDGE('',*,*,#50070,.F.);
#73242=ORIENTED_EDGE('',*,*,#51967,.F.);
#73243=ORIENTED_EDGE('',*,*,#46477,.F.);
#73244=ORIENTED_EDGE('',*,*,#51966,.T.);
#73245=ORIENTED_EDGE('',*,*,#46757,.F.);
#73246=ORIENTED_EDGE('',*,*,#51968,.F.);
#73247=ORIENTED_EDGE('',*,*,#50076,.F.);
#73248=ORIENTED_EDGE('',*,*,#51967,.T.);
#73249=ORIENTED_EDGE('',*,*,#50069,.F.);
#73250=ORIENTED_EDGE('',*,*,#51969,.F.);
#73251=ORIENTED_EDGE('',*,*,#46753,.F.);
#73252=ORIENTED_EDGE('',*,*,#51968,.T.);
#73253=ORIENTED_EDGE('',*,*,#46741,.F.);
#73254=ORIENTED_EDGE('',*,*,#51970,.F.);
#73255=ORIENTED_EDGE('',*,*,#50077,.F.);
#73256=ORIENTED_EDGE('',*,*,#51969,.T.);
#73257=ORIENTED_EDGE('',*,*,#50080,.F.);
#73258=ORIENTED_EDGE('',*,*,#51971,.F.);
#73259=ORIENTED_EDGE('',*,*,#46732,.F.);
#73260=ORIENTED_EDGE('',*,*,#51970,.T.);
#73261=ORIENTED_EDGE('',*,*,#46759,.F.);
#73262=ORIENTED_EDGE('',*,*,#51972,.F.);
#73263=ORIENTED_EDGE('',*,*,#50078,.F.);
#73264=ORIENTED_EDGE('',*,*,#51971,.T.);
#73265=ORIENTED_EDGE('',*,*,#50079,.F.);
#73266=ORIENTED_EDGE('',*,*,#51972,.T.);
#73267=ORIENTED_EDGE('',*,*,#46737,.F.);
#73268=ORIENTED_EDGE('',*,*,#46733,.T.);
#73269=ORIENTED_EDGE('',*,*,#51973,.F.);
#73270=ORIENTED_EDGE('',*,*,#50119,.F.);
#73271=ORIENTED_EDGE('',*,*,#51974,.F.);
#73272=ORIENTED_EDGE('',*,*,#46689,.F.);
#73273=ORIENTED_EDGE('',*,*,#51974,.T.);
#73274=ORIENTED_EDGE('',*,*,#50118,.F.);
#73275=ORIENTED_EDGE('',*,*,#51975,.F.);
#73276=ORIENTED_EDGE('',*,*,#46698,.F.);
#73277=ORIENTED_EDGE('',*,*,#46688,.T.);
#73278=ORIENTED_EDGE('',*,*,#46692,.F.);
#73279=ORIENTED_EDGE('',*,*,#51976,.F.);
#73280=ORIENTED_EDGE('',*,*,#50120,.F.);
#73281=ORIENTED_EDGE('',*,*,#51973,.T.);
#73282=ORIENTED_EDGE('',*,*,#51975,.T.);
#73283=ORIENTED_EDGE('',*,*,#50117,.F.);
#73284=ORIENTED_EDGE('',*,*,#51977,.F.);
#73285=ORIENTED_EDGE('',*,*,#46683,.F.);
#73286=ORIENTED_EDGE('',*,*,#51976,.T.);
#73287=ORIENTED_EDGE('',*,*,#46696,.F.);
#73288=ORIENTED_EDGE('',*,*,#51978,.F.);
#73289=ORIENTED_EDGE('',*,*,#50109,.F.);
#73290=ORIENTED_EDGE('',*,*,#51977,.T.);
#73291=ORIENTED_EDGE('',*,*,#50116,.F.);
#73292=ORIENTED_EDGE('',*,*,#51979,.F.);
#73293=ORIENTED_EDGE('',*,*,#46700,.F.);
#73294=ORIENTED_EDGE('',*,*,#51978,.T.);
#73295=ORIENTED_EDGE('',*,*,#46266,.F.);
#73296=ORIENTED_EDGE('',*,*,#51980,.F.);
#73297=ORIENTED_EDGE('',*,*,#50110,.F.);
#73298=ORIENTED_EDGE('',*,*,#51979,.T.);
#73299=ORIENTED_EDGE('',*,*,#50115,.F.);
#73300=ORIENTED_EDGE('',*,*,#51981,.F.);
#73301=ORIENTED_EDGE('',*,*,#46675,.T.);
#73302=ORIENTED_EDGE('',*,*,#46679,.F.);
#73303=ORIENTED_EDGE('',*,*,#51980,.T.);
#73304=ORIENTED_EDGE('',*,*,#46265,.F.);
#73305=ORIENTED_EDGE('',*,*,#51982,.F.);
#73306=ORIENTED_EDGE('',*,*,#50377,.F.);
#73307=ORIENTED_EDGE('',*,*,#51981,.T.);
#73308=ORIENTED_EDGE('',*,*,#50114,.F.);
#73309=ORIENTED_EDGE('',*,*,#51983,.F.);
#73310=ORIENTED_EDGE('',*,*,#46676,.F.);
#73311=ORIENTED_EDGE('',*,*,#51982,.T.);
#73312=ORIENTED_EDGE('',*,*,#46264,.F.);
#73313=ORIENTED_EDGE('',*,*,#51984,.F.);
#73314=ORIENTED_EDGE('',*,*,#50094,.F.);
#73315=ORIENTED_EDGE('',*,*,#51983,.T.);
#73316=ORIENTED_EDGE('',*,*,#50113,.F.);
#73317=ORIENTED_EDGE('',*,*,#51985,.F.);
#73318=ORIENTED_EDGE('',*,*,#46694,.F.);
#73319=ORIENTED_EDGE('',*,*,#51984,.T.);
#73320=ORIENTED_EDGE('',*,*,#46263,.F.);
#73321=ORIENTED_EDGE('',*,*,#51986,.F.);
#73322=ORIENTED_EDGE('',*,*,#50379,.F.);
#73323=ORIENTED_EDGE('',*,*,#51985,.T.);
#73324=ORIENTED_EDGE('',*,*,#50112,.F.);
#73325=ORIENTED_EDGE('',*,*,#51987,.F.);
#73326=ORIENTED_EDGE('',*,*,#46467,.F.);
#73327=ORIENTED_EDGE('',*,*,#51986,.T.);
#73328=ORIENTED_EDGE('',*,*,#46262,.F.);
#73329=ORIENTED_EDGE('',*,*,#51988,.F.);
#73330=ORIENTED_EDGE('',*,*,#50100,.F.);
#73331=ORIENTED_EDGE('',*,*,#51987,.T.);
#73332=ORIENTED_EDGE('',*,*,#50378,.F.);
#73333=ORIENTED_EDGE('',*,*,#51989,.F.);
#73334=ORIENTED_EDGE('',*,*,#46468,.F.);
#73335=ORIENTED_EDGE('',*,*,#51988,.T.);
#73336=ORIENTED_EDGE('',*,*,#46725,.F.);
#73337=ORIENTED_EDGE('',*,*,#51990,.F.);
#73338=ORIENTED_EDGE('',*,*,#50101,.F.);
#73339=ORIENTED_EDGE('',*,*,#51989,.T.);
#73340=ORIENTED_EDGE('',*,*,#50096,.F.);
#73341=ORIENTED_EDGE('',*,*,#51991,.F.);
#73342=ORIENTED_EDGE('',*,*,#46469,.F.);
#73343=ORIENTED_EDGE('',*,*,#46720,.F.);
#73344=ORIENTED_EDGE('',*,*,#46716,.T.);
#73345=ORIENTED_EDGE('',*,*,#51992,.F.);
#73346=ORIENTED_EDGE('',*,*,#50102,.F.);
#73347=ORIENTED_EDGE('',*,*,#51990,.T.);
#73348=ORIENTED_EDGE('',*,*,#51991,.T.);
#73349=ORIENTED_EDGE('',*,*,#50380,.F.);
#73350=ORIENTED_EDGE('',*,*,#51993,.F.);
#73351=ORIENTED_EDGE('',*,*,#46470,.F.);
#73352=ORIENTED_EDGE('',*,*,#51992,.T.);
#73353=ORIENTED_EDGE('',*,*,#46715,.F.);
#73354=ORIENTED_EDGE('',*,*,#51994,.F.);
#73355=ORIENTED_EDGE('',*,*,#50103,.F.);
#73356=ORIENTED_EDGE('',*,*,#51993,.T.);
#73357=ORIENTED_EDGE('',*,*,#50098,.F.);
#73358=ORIENTED_EDGE('',*,*,#51995,.F.);
#73359=ORIENTED_EDGE('',*,*,#46471,.F.);
#73360=ORIENTED_EDGE('',*,*,#51994,.T.);
#73361=ORIENTED_EDGE('',*,*,#46727,.F.);
#73362=ORIENTED_EDGE('',*,*,#51996,.F.);
#73363=ORIENTED_EDGE('',*,*,#50104,.F.);
#73364=ORIENTED_EDGE('',*,*,#51995,.T.);
#73365=ORIENTED_EDGE('',*,*,#50097,.F.);
#73366=ORIENTED_EDGE('',*,*,#51997,.F.);
#73367=ORIENTED_EDGE('',*,*,#46723,.F.);
#73368=ORIENTED_EDGE('',*,*,#51996,.T.);
#73369=ORIENTED_EDGE('',*,*,#46711,.F.);
#73370=ORIENTED_EDGE('',*,*,#51998,.F.);
#73371=ORIENTED_EDGE('',*,*,#50105,.F.);
#73372=ORIENTED_EDGE('',*,*,#51997,.T.);
#73373=ORIENTED_EDGE('',*,*,#50108,.F.);
#73374=ORIENTED_EDGE('',*,*,#51999,.F.);
#73375=ORIENTED_EDGE('',*,*,#46702,.F.);
#73376=ORIENTED_EDGE('',*,*,#51998,.T.);
#73377=ORIENTED_EDGE('',*,*,#46729,.F.);
#73378=ORIENTED_EDGE('',*,*,#52000,.F.);
#73379=ORIENTED_EDGE('',*,*,#50106,.F.);
#73380=ORIENTED_EDGE('',*,*,#51999,.T.);
#73381=ORIENTED_EDGE('',*,*,#50107,.F.);
#73382=ORIENTED_EDGE('',*,*,#52000,.T.);
#73383=ORIENTED_EDGE('',*,*,#46707,.F.);
#73384=ORIENTED_EDGE('',*,*,#46703,.T.);
#73385=ORIENTED_EDGE('',*,*,#52001,.F.);
#73386=ORIENTED_EDGE('',*,*,#50147,.F.);
#73387=ORIENTED_EDGE('',*,*,#52002,.F.);
#73388=ORIENTED_EDGE('',*,*,#46655,.F.);
#73389=ORIENTED_EDGE('',*,*,#52002,.T.);
#73390=ORIENTED_EDGE('',*,*,#50146,.F.);
#73391=ORIENTED_EDGE('',*,*,#52003,.F.);
#73392=ORIENTED_EDGE('',*,*,#46667,.F.);
#73393=ORIENTED_EDGE('',*,*,#46654,.T.);
#73394=ORIENTED_EDGE('',*,*,#46661,.F.);
#73395=ORIENTED_EDGE('',*,*,#52004,.F.);
#73396=ORIENTED_EDGE('',*,*,#50148,.F.);
#73397=ORIENTED_EDGE('',*,*,#52001,.T.);
#73398=ORIENTED_EDGE('',*,*,#52003,.T.);
#73399=ORIENTED_EDGE('',*,*,#50145,.F.);
#73400=ORIENTED_EDGE('',*,*,#52005,.F.);
#73401=ORIENTED_EDGE('',*,*,#46651,.F.);
#73402=ORIENTED_EDGE('',*,*,#52004,.T.);
#73403=ORIENTED_EDGE('',*,*,#46665,.F.);
#73404=ORIENTED_EDGE('',*,*,#52006,.F.);
#73405=ORIENTED_EDGE('',*,*,#50137,.F.);
#73406=ORIENTED_EDGE('',*,*,#52005,.T.);
#73407=ORIENTED_EDGE('',*,*,#50144,.F.);
#73408=ORIENTED_EDGE('',*,*,#52007,.F.);
#73409=ORIENTED_EDGE('',*,*,#46669,.F.);
#73410=ORIENTED_EDGE('',*,*,#52006,.T.);
#73411=ORIENTED_EDGE('',*,*,#46272,.F.);
#73412=ORIENTED_EDGE('',*,*,#52008,.F.);
#73413=ORIENTED_EDGE('',*,*,#50138,.F.);
#73414=ORIENTED_EDGE('',*,*,#52007,.T.);
#73415=ORIENTED_EDGE('',*,*,#50143,.F.);
#73416=ORIENTED_EDGE('',*,*,#52009,.F.);
#73417=ORIENTED_EDGE('',*,*,#46641,.T.);
#73418=ORIENTED_EDGE('',*,*,#46648,.F.);
#73419=ORIENTED_EDGE('',*,*,#52008,.T.);
#73420=ORIENTED_EDGE('',*,*,#46271,.F.);
#73421=ORIENTED_EDGE('',*,*,#52010,.F.);
#73422=ORIENTED_EDGE('',*,*,#50381,.F.);
#73423=ORIENTED_EDGE('',*,*,#52009,.T.);
#73424=ORIENTED_EDGE('',*,*,#50142,.F.);
#73425=ORIENTED_EDGE('',*,*,#52011,.F.);
#73426=ORIENTED_EDGE('',*,*,#46642,.F.);
#73427=ORIENTED_EDGE('',*,*,#52010,.T.);
#73428=ORIENTED_EDGE('',*,*,#46270,.F.);
#73429=ORIENTED_EDGE('',*,*,#52012,.F.);
#73430=ORIENTED_EDGE('',*,*,#50122,.F.);
#73431=ORIENTED_EDGE('',*,*,#52011,.T.);
#73432=ORIENTED_EDGE('',*,*,#50141,.F.);
#73433=ORIENTED_EDGE('',*,*,#52013,.F.);
#73434=ORIENTED_EDGE('',*,*,#46663,.F.);
#73435=ORIENTED_EDGE('',*,*,#52012,.T.);
#73436=ORIENTED_EDGE('',*,*,#46269,.F.);
#73437=ORIENTED_EDGE('',*,*,#52014,.F.);
#73438=ORIENTED_EDGE('',*,*,#50383,.F.);
#73439=ORIENTED_EDGE('',*,*,#52013,.T.);
#73440=ORIENTED_EDGE('',*,*,#50140,.F.);
#73441=ORIENTED_EDGE('',*,*,#52015,.F.);
#73442=ORIENTED_EDGE('',*,*,#46461,.F.);
#73443=ORIENTED_EDGE('',*,*,#52014,.T.);
#73444=ORIENTED_EDGE('',*,*,#46268,.F.);
#73445=ORIENTED_EDGE('',*,*,#52016,.F.);
#73446=ORIENTED_EDGE('',*,*,#50128,.F.);
#73447=ORIENTED_EDGE('',*,*,#52015,.T.);
#73448=ORIENTED_EDGE('',*,*,#50382,.F.);
#73449=ORIENTED_EDGE('',*,*,#52017,.F.);
#73450=ORIENTED_EDGE('',*,*,#46462,.F.);
#73451=ORIENTED_EDGE('',*,*,#52016,.T.);
#73452=ORIENTED_EDGE('',*,*,#46695,.F.);
#73453=ORIENTED_EDGE('',*,*,#52018,.F.);
#73454=ORIENTED_EDGE('',*,*,#50129,.F.);
#73455=ORIENTED_EDGE('',*,*,#52017,.T.);
#73456=ORIENTED_EDGE('',*,*,#50124,.F.);
#73457=ORIENTED_EDGE('',*,*,#52019,.F.);
#73458=ORIENTED_EDGE('',*,*,#46463,.F.);
#73459=ORIENTED_EDGE('',*,*,#46690,.F.);
#73460=ORIENTED_EDGE('',*,*,#46686,.T.);
#73461=ORIENTED_EDGE('',*,*,#52020,.F.);
#73462=ORIENTED_EDGE('',*,*,#50130,.F.);
#73463=ORIENTED_EDGE('',*,*,#52018,.T.);
#73464=ORIENTED_EDGE('',*,*,#52019,.T.);
#73465=ORIENTED_EDGE('',*,*,#50384,.F.);
#73466=ORIENTED_EDGE('',*,*,#52021,.F.);
#73467=ORIENTED_EDGE('',*,*,#46464,.F.);
#73468=ORIENTED_EDGE('',*,*,#52020,.T.);
#73469=ORIENTED_EDGE('',*,*,#46685,.F.);
#73470=ORIENTED_EDGE('',*,*,#52022,.F.);
#73471=ORIENTED_EDGE('',*,*,#50131,.F.);
#73472=ORIENTED_EDGE('',*,*,#52021,.T.);
#73473=ORIENTED_EDGE('',*,*,#50126,.F.);
#73474=ORIENTED_EDGE('',*,*,#52023,.F.);
#73475=ORIENTED_EDGE('',*,*,#46465,.F.);
#73476=ORIENTED_EDGE('',*,*,#52022,.T.);
#73477=ORIENTED_EDGE('',*,*,#46697,.F.);
#73478=ORIENTED_EDGE('',*,*,#52024,.F.);
#73479=ORIENTED_EDGE('',*,*,#50132,.F.);
#73480=ORIENTED_EDGE('',*,*,#52023,.T.);
#73481=ORIENTED_EDGE('',*,*,#50125,.F.);
#73482=ORIENTED_EDGE('',*,*,#52025,.F.);
#73483=ORIENTED_EDGE('',*,*,#46693,.F.);
#73484=ORIENTED_EDGE('',*,*,#52024,.T.);
#73485=ORIENTED_EDGE('',*,*,#46681,.F.);
#73486=ORIENTED_EDGE('',*,*,#52026,.F.);
#73487=ORIENTED_EDGE('',*,*,#50133,.F.);
#73488=ORIENTED_EDGE('',*,*,#52025,.T.);
#73489=ORIENTED_EDGE('',*,*,#50136,.F.);
#73490=ORIENTED_EDGE('',*,*,#52027,.F.);
#73491=ORIENTED_EDGE('',*,*,#46672,.F.);
#73492=ORIENTED_EDGE('',*,*,#52026,.T.);
#73493=ORIENTED_EDGE('',*,*,#46699,.F.);
#73494=ORIENTED_EDGE('',*,*,#52028,.F.);
#73495=ORIENTED_EDGE('',*,*,#50134,.F.);
#73496=ORIENTED_EDGE('',*,*,#52027,.T.);
#73497=ORIENTED_EDGE('',*,*,#50135,.F.);
#73498=ORIENTED_EDGE('',*,*,#52028,.T.);
#73499=ORIENTED_EDGE('',*,*,#46677,.F.);
#73500=ORIENTED_EDGE('',*,*,#46673,.T.);
#73501=ORIENTED_EDGE('',*,*,#52029,.F.);
#73502=ORIENTED_EDGE('',*,*,#52030,.F.);
#73503=ORIENTED_EDGE('',*,*,#52031,.F.);
#73504=ORIENTED_EDGE('',*,*,#52032,.T.);
#73505=ORIENTED_EDGE('',*,*,#52033,.F.);
#73506=ORIENTED_EDGE('',*,*,#52034,.F.);
#73507=ORIENTED_EDGE('',*,*,#52035,.F.);
#73508=ORIENTED_EDGE('',*,*,#52036,.T.);
#73509=ORIENTED_EDGE('',*,*,#52037,.F.);
#73510=ORIENTED_EDGE('',*,*,#52038,.F.);
#73511=ORIENTED_EDGE('',*,*,#52039,.F.);
#73512=ORIENTED_EDGE('',*,*,#52040,.T.);
#73513=ORIENTED_EDGE('',*,*,#52041,.F.);
#73514=ORIENTED_EDGE('',*,*,#52042,.F.);
#73515=ORIENTED_EDGE('',*,*,#52043,.F.);
#73516=ORIENTED_EDGE('',*,*,#52044,.T.);
#73517=ORIENTED_EDGE('',*,*,#52045,.F.);
#73518=ORIENTED_EDGE('',*,*,#52046,.F.);
#73519=ORIENTED_EDGE('',*,*,#52047,.T.);
#73520=ORIENTED_EDGE('',*,*,#52048,.F.);
#73521=ORIENTED_EDGE('',*,*,#52049,.F.);
#73522=ORIENTED_EDGE('',*,*,#52047,.F.);
#73523=ORIENTED_EDGE('',*,*,#52050,.F.);
#73524=ORIENTED_EDGE('',*,*,#52051,.T.);
#73525=ORIENTED_EDGE('',*,*,#52052,.F.);
#73526=ORIENTED_EDGE('',*,*,#52051,.F.);
#73527=ORIENTED_EDGE('',*,*,#52053,.F.);
#73528=ORIENTED_EDGE('',*,*,#52054,.T.);
#73529=ORIENTED_EDGE('',*,*,#52055,.F.);
#73530=ORIENTED_EDGE('',*,*,#52056,.F.);
#73531=ORIENTED_EDGE('',*,*,#52054,.F.);
#73532=ORIENTED_EDGE('',*,*,#52057,.F.);
#73533=ORIENTED_EDGE('',*,*,#52058,.T.);
#73534=ORIENTED_EDGE('',*,*,#52059,.F.);
#73535=ORIENTED_EDGE('',*,*,#52058,.F.);
#73536=ORIENTED_EDGE('',*,*,#52060,.F.);
#73537=ORIENTED_EDGE('',*,*,#52061,.T.);
#73538=ORIENTED_EDGE('',*,*,#52062,.T.);
#73539=ORIENTED_EDGE('',*,*,#52061,.F.);
#73540=ORIENTED_EDGE('',*,*,#52062,.F.);
#73541=ORIENTED_EDGE('',*,*,#52063,.T.);
#73542=ORIENTED_EDGE('',*,*,#52057,.T.);
#73543=ORIENTED_EDGE('',*,*,#52063,.F.);
#73544=ORIENTED_EDGE('',*,*,#52064,.T.);
#73545=ORIENTED_EDGE('',*,*,#52065,.T.);
#73546=ORIENTED_EDGE('',*,*,#52066,.T.);
#73547=ORIENTED_EDGE('',*,*,#52067,.T.);
#73548=ORIENTED_EDGE('',*,*,#52068,.T.);
#73549=ORIENTED_EDGE('',*,*,#52069,.T.);
#73550=ORIENTED_EDGE('',*,*,#52070,.T.);
#73551=ORIENTED_EDGE('',*,*,#52071,.T.);
#73552=ORIENTED_EDGE('',*,*,#52072,.T.);
#73553=ORIENTED_EDGE('',*,*,#52073,.T.);
#73554=ORIENTED_EDGE('',*,*,#52074,.T.);
#73555=ORIENTED_EDGE('',*,*,#52075,.T.);
#73556=ORIENTED_EDGE('',*,*,#52076,.T.);
#73557=ORIENTED_EDGE('',*,*,#52077,.T.);
#73558=ORIENTED_EDGE('',*,*,#52078,.T.);
#73559=ORIENTED_EDGE('',*,*,#52079,.T.);
#73560=ORIENTED_EDGE('',*,*,#52080,.T.);
#73561=ORIENTED_EDGE('',*,*,#52081,.T.);
#73562=ORIENTED_EDGE('',*,*,#52082,.T.);
#73563=ORIENTED_EDGE('',*,*,#52083,.T.);
#73564=ORIENTED_EDGE('',*,*,#52084,.T.);
#73565=ORIENTED_EDGE('',*,*,#52085,.T.);
#73566=ORIENTED_EDGE('',*,*,#52086,.T.);
#73567=ORIENTED_EDGE('',*,*,#52087,.T.);
#73568=ORIENTED_EDGE('',*,*,#52088,.T.);
#73569=ORIENTED_EDGE('',*,*,#52089,.T.);
#73570=ORIENTED_EDGE('',*,*,#52090,.T.);
#73571=ORIENTED_EDGE('',*,*,#52091,.T.);
#73572=ORIENTED_EDGE('',*,*,#52092,.T.);
#73573=ORIENTED_EDGE('',*,*,#52093,.T.);
#73574=ORIENTED_EDGE('',*,*,#52094,.T.);
#73575=ORIENTED_EDGE('',*,*,#52095,.T.);
#73576=ORIENTED_EDGE('',*,*,#52096,.T.);
#73577=ORIENTED_EDGE('',*,*,#52097,.T.);
#73578=ORIENTED_EDGE('',*,*,#52098,.T.);
#73579=ORIENTED_EDGE('',*,*,#52099,.T.);
#73580=ORIENTED_EDGE('',*,*,#52100,.T.);
#73581=ORIENTED_EDGE('',*,*,#52101,.T.);
#73582=ORIENTED_EDGE('',*,*,#52102,.T.);
#73583=ORIENTED_EDGE('',*,*,#52103,.T.);
#73584=ORIENTED_EDGE('',*,*,#52104,.T.);
#73585=ORIENTED_EDGE('',*,*,#52105,.T.);
#73586=ORIENTED_EDGE('',*,*,#52106,.T.);
#73587=ORIENTED_EDGE('',*,*,#52107,.T.);
#73588=ORIENTED_EDGE('',*,*,#52108,.T.);
#73589=ORIENTED_EDGE('',*,*,#52109,.T.);
#73590=ORIENTED_EDGE('',*,*,#52110,.T.);
#73591=ORIENTED_EDGE('',*,*,#52111,.T.);
#73592=ORIENTED_EDGE('',*,*,#52112,.T.);
#73593=ORIENTED_EDGE('',*,*,#52113,.T.);
#73594=ORIENTED_EDGE('',*,*,#52114,.T.);
#73595=ORIENTED_EDGE('',*,*,#52115,.T.);
#73596=ORIENTED_EDGE('',*,*,#52116,.T.);
#73597=ORIENTED_EDGE('',*,*,#52117,.T.);
#73598=ORIENTED_EDGE('',*,*,#52118,.T.);
#73599=ORIENTED_EDGE('',*,*,#52119,.T.);
#73600=ORIENTED_EDGE('',*,*,#52120,.T.);
#73601=ORIENTED_EDGE('',*,*,#52121,.T.);
#73602=ORIENTED_EDGE('',*,*,#52122,.T.);
#73603=ORIENTED_EDGE('',*,*,#52123,.T.);
#73604=ORIENTED_EDGE('',*,*,#52124,.T.);
#73605=ORIENTED_EDGE('',*,*,#52125,.T.);
#73606=ORIENTED_EDGE('',*,*,#52126,.T.);
#73607=ORIENTED_EDGE('',*,*,#52127,.T.);
#73608=ORIENTED_EDGE('',*,*,#52128,.T.);
#73609=ORIENTED_EDGE('',*,*,#52129,.T.);
#73610=ORIENTED_EDGE('',*,*,#52130,.T.);
#73611=ORIENTED_EDGE('',*,*,#52131,.T.);
#73612=ORIENTED_EDGE('',*,*,#52132,.T.);
#73613=ORIENTED_EDGE('',*,*,#52133,.T.);
#73614=ORIENTED_EDGE('',*,*,#52134,.T.);
#73615=ORIENTED_EDGE('',*,*,#52135,.T.);
#73616=ORIENTED_EDGE('',*,*,#52136,.T.);
#73617=ORIENTED_EDGE('',*,*,#52137,.T.);
#73618=ORIENTED_EDGE('',*,*,#52138,.T.);
#73619=ORIENTED_EDGE('',*,*,#52139,.T.);
#73620=ORIENTED_EDGE('',*,*,#52140,.T.);
#73621=ORIENTED_EDGE('',*,*,#52141,.T.);
#73622=ORIENTED_EDGE('',*,*,#52142,.T.);
#73623=ORIENTED_EDGE('',*,*,#52143,.T.);
#73624=ORIENTED_EDGE('',*,*,#52144,.T.);
#73625=ORIENTED_EDGE('',*,*,#52145,.T.);
#73626=ORIENTED_EDGE('',*,*,#52146,.T.);
#73627=ORIENTED_EDGE('',*,*,#52147,.T.);
#73628=ORIENTED_EDGE('',*,*,#52148,.T.);
#73629=ORIENTED_EDGE('',*,*,#52149,.T.);
#73630=ORIENTED_EDGE('',*,*,#52150,.T.);
#73631=ORIENTED_EDGE('',*,*,#52151,.T.);
#73632=ORIENTED_EDGE('',*,*,#52152,.T.);
#73633=ORIENTED_EDGE('',*,*,#52153,.T.);
#73634=ORIENTED_EDGE('',*,*,#52154,.T.);
#73635=ORIENTED_EDGE('',*,*,#52155,.T.);
#73636=ORIENTED_EDGE('',*,*,#52156,.T.);
#73637=ORIENTED_EDGE('',*,*,#52157,.T.);
#73638=ORIENTED_EDGE('',*,*,#52158,.T.);
#73639=ORIENTED_EDGE('',*,*,#52159,.T.);
#73640=ORIENTED_EDGE('',*,*,#52160,.T.);
#73641=ORIENTED_EDGE('',*,*,#52161,.T.);
#73642=ORIENTED_EDGE('',*,*,#52162,.T.);
#73643=ORIENTED_EDGE('',*,*,#52163,.T.);
#73644=ORIENTED_EDGE('',*,*,#52164,.T.);
#73645=ORIENTED_EDGE('',*,*,#52165,.T.);
#73646=ORIENTED_EDGE('',*,*,#52166,.T.);
#73647=ORIENTED_EDGE('',*,*,#52167,.T.);
#73648=ORIENTED_EDGE('',*,*,#52168,.T.);
#73649=ORIENTED_EDGE('',*,*,#52169,.T.);
#73650=ORIENTED_EDGE('',*,*,#52170,.T.);
#73651=ORIENTED_EDGE('',*,*,#52171,.T.);
#73652=ORIENTED_EDGE('',*,*,#52172,.T.);
#73653=ORIENTED_EDGE('',*,*,#52173,.T.);
#73654=ORIENTED_EDGE('',*,*,#52174,.T.);
#73655=ORIENTED_EDGE('',*,*,#52175,.T.);
#73656=ORIENTED_EDGE('',*,*,#52176,.T.);
#73657=ORIENTED_EDGE('',*,*,#52177,.T.);
#73658=ORIENTED_EDGE('',*,*,#52178,.T.);
#73659=ORIENTED_EDGE('',*,*,#52179,.T.);
#73660=ORIENTED_EDGE('',*,*,#52180,.T.);
#73661=ORIENTED_EDGE('',*,*,#52181,.T.);
#73662=ORIENTED_EDGE('',*,*,#52182,.T.);
#73663=ORIENTED_EDGE('',*,*,#52183,.T.);
#73664=ORIENTED_EDGE('',*,*,#52184,.T.);
#73665=ORIENTED_EDGE('',*,*,#52185,.T.);
#73666=ORIENTED_EDGE('',*,*,#52186,.T.);
#73667=ORIENTED_EDGE('',*,*,#52187,.T.);
#73668=ORIENTED_EDGE('',*,*,#52188,.T.);
#73669=ORIENTED_EDGE('',*,*,#52189,.T.);
#73670=ORIENTED_EDGE('',*,*,#52190,.T.);
#73671=ORIENTED_EDGE('',*,*,#52191,.T.);
#73672=ORIENTED_EDGE('',*,*,#52192,.T.);
#73673=ORIENTED_EDGE('',*,*,#52193,.T.);
#73674=ORIENTED_EDGE('',*,*,#52194,.T.);
#73675=ORIENTED_EDGE('',*,*,#52195,.T.);
#73676=ORIENTED_EDGE('',*,*,#52196,.T.);
#73677=ORIENTED_EDGE('',*,*,#52197,.T.);
#73678=ORIENTED_EDGE('',*,*,#52198,.T.);
#73679=ORIENTED_EDGE('',*,*,#52199,.T.);
#73680=ORIENTED_EDGE('',*,*,#52200,.T.);
#73681=ORIENTED_EDGE('',*,*,#52201,.T.);
#73682=ORIENTED_EDGE('',*,*,#52202,.T.);
#73683=ORIENTED_EDGE('',*,*,#52203,.T.);
#73684=ORIENTED_EDGE('',*,*,#52204,.T.);
#73685=ORIENTED_EDGE('',*,*,#52205,.T.);
#73686=ORIENTED_EDGE('',*,*,#52206,.T.);
#73687=ORIENTED_EDGE('',*,*,#52207,.T.);
#73688=ORIENTED_EDGE('',*,*,#52208,.T.);
#73689=ORIENTED_EDGE('',*,*,#52209,.T.);
#73690=ORIENTED_EDGE('',*,*,#52210,.T.);
#73691=ORIENTED_EDGE('',*,*,#52211,.T.);
#73692=ORIENTED_EDGE('',*,*,#52212,.T.);
#73693=ORIENTED_EDGE('',*,*,#52213,.T.);
#73694=ORIENTED_EDGE('',*,*,#52214,.T.);
#73695=ORIENTED_EDGE('',*,*,#52215,.T.);
#73696=ORIENTED_EDGE('',*,*,#52216,.T.);
#73697=ORIENTED_EDGE('',*,*,#52217,.T.);
#73698=ORIENTED_EDGE('',*,*,#52218,.T.);
#73699=ORIENTED_EDGE('',*,*,#52219,.T.);
#73700=ORIENTED_EDGE('',*,*,#52220,.T.);
#73701=ORIENTED_EDGE('',*,*,#52221,.T.);
#73702=ORIENTED_EDGE('',*,*,#52222,.T.);
#73703=ORIENTED_EDGE('',*,*,#52223,.T.);
#73704=ORIENTED_EDGE('',*,*,#52224,.T.);
#73705=ORIENTED_EDGE('',*,*,#52225,.T.);
#73706=ORIENTED_EDGE('',*,*,#52226,.T.);
#73707=ORIENTED_EDGE('',*,*,#52227,.T.);
#73708=ORIENTED_EDGE('',*,*,#52228,.T.);
#73709=ORIENTED_EDGE('',*,*,#52229,.T.);
#73710=ORIENTED_EDGE('',*,*,#52230,.T.);
#73711=ORIENTED_EDGE('',*,*,#52231,.T.);
#73712=ORIENTED_EDGE('',*,*,#52232,.T.);
#73713=ORIENTED_EDGE('',*,*,#52233,.T.);
#73714=ORIENTED_EDGE('',*,*,#52234,.T.);
#73715=ORIENTED_EDGE('',*,*,#52235,.T.);
#73716=ORIENTED_EDGE('',*,*,#52236,.T.);
#73717=ORIENTED_EDGE('',*,*,#52237,.T.);
#73718=ORIENTED_EDGE('',*,*,#52238,.T.);
#73719=ORIENTED_EDGE('',*,*,#52239,.T.);
#73720=ORIENTED_EDGE('',*,*,#52240,.T.);
#73721=ORIENTED_EDGE('',*,*,#52241,.T.);
#73722=ORIENTED_EDGE('',*,*,#52242,.T.);
#73723=ORIENTED_EDGE('',*,*,#52243,.T.);
#73724=ORIENTED_EDGE('',*,*,#52041,.T.);
#73725=ORIENTED_EDGE('',*,*,#52244,.T.);
#73726=ORIENTED_EDGE('',*,*,#52055,.T.);
#73727=ORIENTED_EDGE('',*,*,#52056,.T.);
#73728=ORIENTED_EDGE('',*,*,#52244,.F.);
#73729=ORIENTED_EDGE('',*,*,#52045,.T.);
#73730=ORIENTED_EDGE('',*,*,#52245,.T.);
#73731=ORIENTED_EDGE('',*,*,#52246,.T.);
#73732=ORIENTED_EDGE('',*,*,#52247,.T.);
#73733=ORIENTED_EDGE('',*,*,#52248,.T.);
#73734=ORIENTED_EDGE('',*,*,#52249,.T.);
#73735=ORIENTED_EDGE('',*,*,#52250,.T.);
#73736=ORIENTED_EDGE('',*,*,#52251,.T.);
#73737=ORIENTED_EDGE('',*,*,#52252,.T.);
#73738=ORIENTED_EDGE('',*,*,#52253,.T.);
#73739=ORIENTED_EDGE('',*,*,#52254,.T.);
#73740=ORIENTED_EDGE('',*,*,#52255,.T.);
#73741=ORIENTED_EDGE('',*,*,#52256,.T.);
#73742=ORIENTED_EDGE('',*,*,#52257,.T.);
#73743=ORIENTED_EDGE('',*,*,#52258,.T.);
#73744=ORIENTED_EDGE('',*,*,#52259,.T.);
#73745=ORIENTED_EDGE('',*,*,#52260,.T.);
#73746=ORIENTED_EDGE('',*,*,#52261,.T.);
#73747=ORIENTED_EDGE('',*,*,#52262,.T.);
#73748=ORIENTED_EDGE('',*,*,#52263,.T.);
#73749=ORIENTED_EDGE('',*,*,#52264,.T.);
#73750=ORIENTED_EDGE('',*,*,#52265,.T.);
#73751=ORIENTED_EDGE('',*,*,#52266,.T.);
#73752=ORIENTED_EDGE('',*,*,#52267,.T.);
#73753=ORIENTED_EDGE('',*,*,#52268,.T.);
#73754=ORIENTED_EDGE('',*,*,#52269,.T.);
#73755=ORIENTED_EDGE('',*,*,#52270,.T.);
#73756=ORIENTED_EDGE('',*,*,#52271,.T.);
#73757=ORIENTED_EDGE('',*,*,#52272,.T.);
#73758=ORIENTED_EDGE('',*,*,#52273,.T.);
#73759=ORIENTED_EDGE('',*,*,#52274,.T.);
#73760=ORIENTED_EDGE('',*,*,#52275,.T.);
#73761=ORIENTED_EDGE('',*,*,#52276,.T.);
#73762=ORIENTED_EDGE('',*,*,#52277,.T.);
#73763=ORIENTED_EDGE('',*,*,#52278,.T.);
#73764=ORIENTED_EDGE('',*,*,#52279,.T.);
#73765=ORIENTED_EDGE('',*,*,#52280,.T.);
#73766=ORIENTED_EDGE('',*,*,#52281,.T.);
#73767=ORIENTED_EDGE('',*,*,#52282,.T.);
#73768=ORIENTED_EDGE('',*,*,#52283,.T.);
#73769=ORIENTED_EDGE('',*,*,#52284,.T.);
#73770=ORIENTED_EDGE('',*,*,#52285,.T.);
#73771=ORIENTED_EDGE('',*,*,#52286,.T.);
#73772=ORIENTED_EDGE('',*,*,#52287,.T.);
#73773=ORIENTED_EDGE('',*,*,#52288,.T.);
#73774=ORIENTED_EDGE('',*,*,#52289,.T.);
#73775=ORIENTED_EDGE('',*,*,#52290,.T.);
#73776=ORIENTED_EDGE('',*,*,#52291,.T.);
#73777=ORIENTED_EDGE('',*,*,#52292,.T.);
#73778=ORIENTED_EDGE('',*,*,#52293,.T.);
#73779=ORIENTED_EDGE('',*,*,#52294,.T.);
#73780=ORIENTED_EDGE('',*,*,#52295,.T.);
#73781=ORIENTED_EDGE('',*,*,#52296,.T.);
#73782=ORIENTED_EDGE('',*,*,#52297,.T.);
#73783=ORIENTED_EDGE('',*,*,#52298,.T.);
#73784=ORIENTED_EDGE('',*,*,#52299,.T.);
#73785=ORIENTED_EDGE('',*,*,#52300,.T.);
#73786=ORIENTED_EDGE('',*,*,#52301,.T.);
#73787=ORIENTED_EDGE('',*,*,#52302,.T.);
#73788=ORIENTED_EDGE('',*,*,#52303,.T.);
#73789=ORIENTED_EDGE('',*,*,#52304,.T.);
#73790=ORIENTED_EDGE('',*,*,#52305,.T.);
#73791=ORIENTED_EDGE('',*,*,#52306,.T.);
#73792=ORIENTED_EDGE('',*,*,#52307,.T.);
#73793=ORIENTED_EDGE('',*,*,#52308,.T.);
#73794=ORIENTED_EDGE('',*,*,#52309,.T.);
#73795=ORIENTED_EDGE('',*,*,#52310,.T.);
#73796=ORIENTED_EDGE('',*,*,#52311,.T.);
#73797=ORIENTED_EDGE('',*,*,#52312,.T.);
#73798=ORIENTED_EDGE('',*,*,#52313,.T.);
#73799=ORIENTED_EDGE('',*,*,#52314,.T.);
#73800=ORIENTED_EDGE('',*,*,#52315,.T.);
#73801=ORIENTED_EDGE('',*,*,#52316,.T.);
#73802=ORIENTED_EDGE('',*,*,#52317,.T.);
#73803=ORIENTED_EDGE('',*,*,#52318,.T.);
#73804=ORIENTED_EDGE('',*,*,#52319,.T.);
#73805=ORIENTED_EDGE('',*,*,#52320,.T.);
#73806=ORIENTED_EDGE('',*,*,#52321,.T.);
#73807=ORIENTED_EDGE('',*,*,#52322,.T.);
#73808=ORIENTED_EDGE('',*,*,#52323,.T.);
#73809=ORIENTED_EDGE('',*,*,#52324,.T.);
#73810=ORIENTED_EDGE('',*,*,#52325,.T.);
#73811=ORIENTED_EDGE('',*,*,#52326,.T.);
#73812=ORIENTED_EDGE('',*,*,#52327,.T.);
#73813=ORIENTED_EDGE('',*,*,#52328,.T.);
#73814=ORIENTED_EDGE('',*,*,#52329,.T.);
#73815=ORIENTED_EDGE('',*,*,#52330,.T.);
#73816=ORIENTED_EDGE('',*,*,#52331,.T.);
#73817=ORIENTED_EDGE('',*,*,#52332,.T.);
#73818=ORIENTED_EDGE('',*,*,#52333,.T.);
#73819=ORIENTED_EDGE('',*,*,#52033,.T.);
#73820=ORIENTED_EDGE('',*,*,#52334,.T.);
#73821=ORIENTED_EDGE('',*,*,#52335,.T.);
#73822=ORIENTED_EDGE('',*,*,#52336,.T.);
#73823=ORIENTED_EDGE('',*,*,#52337,.T.);
#73824=ORIENTED_EDGE('',*,*,#52338,.T.);
#73825=ORIENTED_EDGE('',*,*,#52339,.T.);
#73826=ORIENTED_EDGE('',*,*,#52340,.T.);
#73827=ORIENTED_EDGE('',*,*,#52341,.T.);
#73828=ORIENTED_EDGE('',*,*,#52342,.T.);
#73829=ORIENTED_EDGE('',*,*,#52343,.T.);
#73830=ORIENTED_EDGE('',*,*,#52344,.T.);
#73831=ORIENTED_EDGE('',*,*,#52345,.T.);
#73832=ORIENTED_EDGE('',*,*,#52346,.T.);
#73833=ORIENTED_EDGE('',*,*,#52347,.T.);
#73834=ORIENTED_EDGE('',*,*,#52348,.T.);
#73835=ORIENTED_EDGE('',*,*,#52349,.T.);
#73836=ORIENTED_EDGE('',*,*,#52350,.T.);
#73837=ORIENTED_EDGE('',*,*,#52351,.T.);
#73838=ORIENTED_EDGE('',*,*,#52352,.T.);
#73839=ORIENTED_EDGE('',*,*,#52353,.T.);
#73840=ORIENTED_EDGE('',*,*,#52354,.T.);
#73841=ORIENTED_EDGE('',*,*,#52355,.T.);
#73842=ORIENTED_EDGE('',*,*,#52356,.T.);
#73843=ORIENTED_EDGE('',*,*,#52357,.T.);
#73844=ORIENTED_EDGE('',*,*,#52358,.T.);
#73845=ORIENTED_EDGE('',*,*,#52359,.T.);
#73846=ORIENTED_EDGE('',*,*,#52360,.T.);
#73847=ORIENTED_EDGE('',*,*,#52361,.T.);
#73848=ORIENTED_EDGE('',*,*,#52362,.T.);
#73849=ORIENTED_EDGE('',*,*,#52363,.T.);
#73850=ORIENTED_EDGE('',*,*,#52364,.T.);
#73851=ORIENTED_EDGE('',*,*,#52365,.T.);
#73852=ORIENTED_EDGE('',*,*,#52366,.T.);
#73853=ORIENTED_EDGE('',*,*,#52367,.T.);
#73854=ORIENTED_EDGE('',*,*,#52368,.T.);
#73855=ORIENTED_EDGE('',*,*,#52369,.T.);
#73856=ORIENTED_EDGE('',*,*,#52370,.T.);
#73857=ORIENTED_EDGE('',*,*,#52371,.T.);
#73858=ORIENTED_EDGE('',*,*,#52372,.T.);
#73859=ORIENTED_EDGE('',*,*,#52373,.T.);
#73860=ORIENTED_EDGE('',*,*,#52374,.T.);
#73861=ORIENTED_EDGE('',*,*,#52375,.T.);
#73862=ORIENTED_EDGE('',*,*,#52376,.T.);
#73863=ORIENTED_EDGE('',*,*,#52377,.T.);
#73864=ORIENTED_EDGE('',*,*,#52378,.T.);
#73865=ORIENTED_EDGE('',*,*,#52379,.T.);
#73866=ORIENTED_EDGE('',*,*,#52380,.T.);
#73867=ORIENTED_EDGE('',*,*,#52381,.T.);
#73868=ORIENTED_EDGE('',*,*,#52382,.T.);
#73869=ORIENTED_EDGE('',*,*,#52383,.T.);
#73870=ORIENTED_EDGE('',*,*,#52384,.T.);
#73871=ORIENTED_EDGE('',*,*,#52385,.T.);
#73872=ORIENTED_EDGE('',*,*,#52386,.T.);
#73873=ORIENTED_EDGE('',*,*,#52387,.T.);
#73874=ORIENTED_EDGE('',*,*,#52388,.T.);
#73875=ORIENTED_EDGE('',*,*,#52389,.T.);
#73876=ORIENTED_EDGE('',*,*,#52390,.T.);
#73877=ORIENTED_EDGE('',*,*,#52391,.T.);
#73878=ORIENTED_EDGE('',*,*,#52392,.T.);
#73879=ORIENTED_EDGE('',*,*,#52393,.T.);
#73880=ORIENTED_EDGE('',*,*,#52394,.T.);
#73881=ORIENTED_EDGE('',*,*,#52395,.T.);
#73882=ORIENTED_EDGE('',*,*,#52396,.T.);
#73883=ORIENTED_EDGE('',*,*,#52397,.T.);
#73884=ORIENTED_EDGE('',*,*,#52398,.T.);
#73885=ORIENTED_EDGE('',*,*,#52399,.T.);
#73886=ORIENTED_EDGE('',*,*,#52400,.T.);
#73887=ORIENTED_EDGE('',*,*,#52401,.T.);
#73888=ORIENTED_EDGE('',*,*,#52402,.T.);
#73889=ORIENTED_EDGE('',*,*,#52403,.T.);
#73890=ORIENTED_EDGE('',*,*,#52404,.T.);
#73891=ORIENTED_EDGE('',*,*,#52405,.T.);
#73892=ORIENTED_EDGE('',*,*,#52406,.T.);
#73893=ORIENTED_EDGE('',*,*,#52407,.T.);
#73894=ORIENTED_EDGE('',*,*,#52408,.T.);
#73895=ORIENTED_EDGE('',*,*,#52409,.T.);
#73896=ORIENTED_EDGE('',*,*,#52410,.T.);
#73897=ORIENTED_EDGE('',*,*,#52411,.T.);
#73898=ORIENTED_EDGE('',*,*,#52412,.T.);
#73899=ORIENTED_EDGE('',*,*,#52413,.T.);
#73900=ORIENTED_EDGE('',*,*,#52414,.T.);
#73901=ORIENTED_EDGE('',*,*,#52415,.T.);
#73902=ORIENTED_EDGE('',*,*,#52416,.T.);
#73903=ORIENTED_EDGE('',*,*,#52417,.T.);
#73904=ORIENTED_EDGE('',*,*,#52418,.T.);
#73905=ORIENTED_EDGE('',*,*,#52419,.T.);
#73906=ORIENTED_EDGE('',*,*,#52420,.T.);
#73907=ORIENTED_EDGE('',*,*,#52421,.T.);
#73908=ORIENTED_EDGE('',*,*,#52422,.T.);
#73909=ORIENTED_EDGE('',*,*,#52039,.T.);
#73910=ORIENTED_EDGE('',*,*,#52423,.T.);
#73911=ORIENTED_EDGE('',*,*,#52424,.T.);
#73912=ORIENTED_EDGE('',*,*,#52425,.T.);
#73913=ORIENTED_EDGE('',*,*,#52426,.T.);
#73914=ORIENTED_EDGE('',*,*,#52427,.T.);
#73915=ORIENTED_EDGE('',*,*,#52428,.T.);
#73916=ORIENTED_EDGE('',*,*,#52429,.T.);
#73917=ORIENTED_EDGE('',*,*,#52430,.T.);
#73918=ORIENTED_EDGE('',*,*,#52431,.T.);
#73919=ORIENTED_EDGE('',*,*,#52432,.T.);
#73920=ORIENTED_EDGE('',*,*,#52433,.T.);
#73921=ORIENTED_EDGE('',*,*,#52434,.T.);
#73922=ORIENTED_EDGE('',*,*,#52435,.T.);
#73923=ORIENTED_EDGE('',*,*,#52436,.T.);
#73924=ORIENTED_EDGE('',*,*,#52437,.T.);
#73925=ORIENTED_EDGE('',*,*,#52438,.T.);
#73926=ORIENTED_EDGE('',*,*,#52439,.T.);
#73927=ORIENTED_EDGE('',*,*,#52440,.T.);
#73928=ORIENTED_EDGE('',*,*,#52441,.T.);
#73929=ORIENTED_EDGE('',*,*,#52442,.T.);
#73930=ORIENTED_EDGE('',*,*,#52443,.T.);
#73931=ORIENTED_EDGE('',*,*,#52444,.T.);
#73932=ORIENTED_EDGE('',*,*,#52445,.T.);
#73933=ORIENTED_EDGE('',*,*,#52446,.T.);
#73934=ORIENTED_EDGE('',*,*,#52447,.T.);
#73935=ORIENTED_EDGE('',*,*,#52448,.T.);
#73936=ORIENTED_EDGE('',*,*,#52449,.T.);
#73937=ORIENTED_EDGE('',*,*,#52450,.T.);
#73938=ORIENTED_EDGE('',*,*,#52451,.T.);
#73939=ORIENTED_EDGE('',*,*,#52452,.T.);
#73940=ORIENTED_EDGE('',*,*,#52453,.T.);
#73941=ORIENTED_EDGE('',*,*,#52454,.T.);
#73942=ORIENTED_EDGE('',*,*,#52455,.T.);
#73943=ORIENTED_EDGE('',*,*,#52456,.T.);
#73944=ORIENTED_EDGE('',*,*,#52457,.T.);
#73945=ORIENTED_EDGE('',*,*,#52458,.T.);
#73946=ORIENTED_EDGE('',*,*,#52459,.T.);
#73947=ORIENTED_EDGE('',*,*,#52460,.T.);
#73948=ORIENTED_EDGE('',*,*,#52461,.T.);
#73949=ORIENTED_EDGE('',*,*,#52462,.T.);
#73950=ORIENTED_EDGE('',*,*,#52463,.T.);
#73951=ORIENTED_EDGE('',*,*,#52464,.T.);
#73952=ORIENTED_EDGE('',*,*,#52465,.T.);
#73953=ORIENTED_EDGE('',*,*,#52466,.T.);
#73954=ORIENTED_EDGE('',*,*,#52467,.T.);
#73955=ORIENTED_EDGE('',*,*,#52468,.T.);
#73956=ORIENTED_EDGE('',*,*,#52469,.T.);
#73957=ORIENTED_EDGE('',*,*,#52470,.T.);
#73958=ORIENTED_EDGE('',*,*,#52471,.T.);
#73959=ORIENTED_EDGE('',*,*,#52472,.T.);
#73960=ORIENTED_EDGE('',*,*,#52473,.T.);
#73961=ORIENTED_EDGE('',*,*,#52474,.T.);
#73962=ORIENTED_EDGE('',*,*,#52475,.T.);
#73963=ORIENTED_EDGE('',*,*,#52476,.T.);
#73964=ORIENTED_EDGE('',*,*,#52477,.T.);
#73965=ORIENTED_EDGE('',*,*,#52478,.T.);
#73966=ORIENTED_EDGE('',*,*,#52479,.T.);
#73967=ORIENTED_EDGE('',*,*,#52480,.T.);
#73968=ORIENTED_EDGE('',*,*,#52481,.T.);
#73969=ORIENTED_EDGE('',*,*,#52482,.T.);
#73970=ORIENTED_EDGE('',*,*,#52483,.T.);
#73971=ORIENTED_EDGE('',*,*,#52484,.T.);
#73972=ORIENTED_EDGE('',*,*,#52485,.T.);
#73973=ORIENTED_EDGE('',*,*,#52486,.T.);
#73974=ORIENTED_EDGE('',*,*,#52487,.T.);
#73975=ORIENTED_EDGE('',*,*,#52488,.T.);
#73976=ORIENTED_EDGE('',*,*,#52489,.T.);
#73977=ORIENTED_EDGE('',*,*,#52490,.T.);
#73978=ORIENTED_EDGE('',*,*,#52491,.T.);
#73979=ORIENTED_EDGE('',*,*,#52492,.T.);
#73980=ORIENTED_EDGE('',*,*,#52493,.T.);
#73981=ORIENTED_EDGE('',*,*,#52494,.T.);
#73982=ORIENTED_EDGE('',*,*,#52495,.T.);
#73983=ORIENTED_EDGE('',*,*,#52496,.T.);
#73984=ORIENTED_EDGE('',*,*,#52497,.T.);
#73985=ORIENTED_EDGE('',*,*,#52498,.T.);
#73986=ORIENTED_EDGE('',*,*,#52499,.T.);
#73987=ORIENTED_EDGE('',*,*,#52500,.T.);
#73988=ORIENTED_EDGE('',*,*,#52501,.T.);
#73989=ORIENTED_EDGE('',*,*,#52502,.T.);
#73990=ORIENTED_EDGE('',*,*,#52503,.T.);
#73991=ORIENTED_EDGE('',*,*,#52504,.T.);
#73992=ORIENTED_EDGE('',*,*,#52505,.T.);
#73993=ORIENTED_EDGE('',*,*,#52506,.T.);
#73994=ORIENTED_EDGE('',*,*,#52507,.T.);
#73995=ORIENTED_EDGE('',*,*,#52508,.T.);
#73996=ORIENTED_EDGE('',*,*,#52509,.T.);
#73997=ORIENTED_EDGE('',*,*,#52510,.T.);
#73998=ORIENTED_EDGE('',*,*,#52511,.T.);
#73999=ORIENTED_EDGE('',*,*,#52512,.T.);
#74000=ORIENTED_EDGE('',*,*,#52513,.T.);
#74001=ORIENTED_EDGE('',*,*,#52514,.T.);
#74002=ORIENTED_EDGE('',*,*,#52515,.T.);
#74003=ORIENTED_EDGE('',*,*,#52516,.T.);
#74004=ORIENTED_EDGE('',*,*,#52517,.T.);
#74005=ORIENTED_EDGE('',*,*,#52518,.T.);
#74006=ORIENTED_EDGE('',*,*,#52519,.T.);
#74007=ORIENTED_EDGE('',*,*,#52520,.T.);
#74008=ORIENTED_EDGE('',*,*,#52521,.T.);
#74009=ORIENTED_EDGE('',*,*,#52522,.T.);
#74010=ORIENTED_EDGE('',*,*,#52523,.T.);
#74011=ORIENTED_EDGE('',*,*,#52524,.T.);
#74012=ORIENTED_EDGE('',*,*,#52525,.T.);
#74013=ORIENTED_EDGE('',*,*,#52526,.T.);
#74014=ORIENTED_EDGE('',*,*,#52527,.T.);
#74015=ORIENTED_EDGE('',*,*,#52528,.T.);
#74016=ORIENTED_EDGE('',*,*,#52529,.T.);
#74017=ORIENTED_EDGE('',*,*,#52530,.T.);
#74018=ORIENTED_EDGE('',*,*,#52531,.T.);
#74019=ORIENTED_EDGE('',*,*,#52532,.T.);
#74020=ORIENTED_EDGE('',*,*,#52533,.T.);
#74021=ORIENTED_EDGE('',*,*,#52534,.T.);
#74022=ORIENTED_EDGE('',*,*,#52535,.T.);
#74023=ORIENTED_EDGE('',*,*,#52536,.T.);
#74024=ORIENTED_EDGE('',*,*,#52537,.T.);
#74025=ORIENTED_EDGE('',*,*,#52538,.T.);
#74026=ORIENTED_EDGE('',*,*,#52539,.T.);
#74027=ORIENTED_EDGE('',*,*,#52540,.T.);
#74028=ORIENTED_EDGE('',*,*,#52541,.T.);
#74029=ORIENTED_EDGE('',*,*,#52542,.T.);
#74030=ORIENTED_EDGE('',*,*,#52543,.T.);
#74031=ORIENTED_EDGE('',*,*,#52544,.T.);
#74032=ORIENTED_EDGE('',*,*,#52545,.T.);
#74033=ORIENTED_EDGE('',*,*,#52546,.T.);
#74034=ORIENTED_EDGE('',*,*,#52547,.T.);
#74035=ORIENTED_EDGE('',*,*,#52548,.T.);
#74036=ORIENTED_EDGE('',*,*,#52549,.T.);
#74037=ORIENTED_EDGE('',*,*,#52550,.T.);
#74038=ORIENTED_EDGE('',*,*,#52551,.T.);
#74039=ORIENTED_EDGE('',*,*,#52552,.T.);
#74040=ORIENTED_EDGE('',*,*,#52553,.T.);
#74041=ORIENTED_EDGE('',*,*,#52554,.T.);
#74042=ORIENTED_EDGE('',*,*,#52555,.T.);
#74043=ORIENTED_EDGE('',*,*,#52556,.T.);
#74044=ORIENTED_EDGE('',*,*,#52557,.T.);
#74045=ORIENTED_EDGE('',*,*,#52558,.T.);
#74046=ORIENTED_EDGE('',*,*,#52559,.T.);
#74047=ORIENTED_EDGE('',*,*,#52560,.T.);
#74048=ORIENTED_EDGE('',*,*,#52561,.T.);
#74049=ORIENTED_EDGE('',*,*,#52562,.T.);
#74050=ORIENTED_EDGE('',*,*,#52563,.T.);
#74051=ORIENTED_EDGE('',*,*,#52564,.T.);
#74052=ORIENTED_EDGE('',*,*,#52565,.T.);
#74053=ORIENTED_EDGE('',*,*,#52566,.T.);
#74054=ORIENTED_EDGE('',*,*,#52567,.T.);
#74055=ORIENTED_EDGE('',*,*,#52568,.T.);
#74056=ORIENTED_EDGE('',*,*,#52569,.T.);
#74057=ORIENTED_EDGE('',*,*,#52570,.T.);
#74058=ORIENTED_EDGE('',*,*,#52571,.T.);
#74059=ORIENTED_EDGE('',*,*,#52572,.T.);
#74060=ORIENTED_EDGE('',*,*,#52573,.T.);
#74061=ORIENTED_EDGE('',*,*,#52574,.T.);
#74062=ORIENTED_EDGE('',*,*,#52575,.T.);
#74063=ORIENTED_EDGE('',*,*,#52576,.T.);
#74064=ORIENTED_EDGE('',*,*,#52577,.T.);
#74065=ORIENTED_EDGE('',*,*,#52578,.T.);
#74066=ORIENTED_EDGE('',*,*,#52579,.T.);
#74067=ORIENTED_EDGE('',*,*,#52580,.T.);
#74068=ORIENTED_EDGE('',*,*,#52581,.T.);
#74069=ORIENTED_EDGE('',*,*,#52582,.T.);
#74070=ORIENTED_EDGE('',*,*,#52583,.T.);
#74071=ORIENTED_EDGE('',*,*,#52584,.T.);
#74072=ORIENTED_EDGE('',*,*,#52585,.T.);
#74073=ORIENTED_EDGE('',*,*,#52586,.T.);
#74074=ORIENTED_EDGE('',*,*,#52587,.T.);
#74075=ORIENTED_EDGE('',*,*,#52588,.T.);
#74076=ORIENTED_EDGE('',*,*,#52589,.T.);
#74077=ORIENTED_EDGE('',*,*,#52590,.T.);
#74078=ORIENTED_EDGE('',*,*,#52591,.T.);
#74079=ORIENTED_EDGE('',*,*,#52592,.T.);
#74080=ORIENTED_EDGE('',*,*,#52593,.T.);
#74081=ORIENTED_EDGE('',*,*,#52594,.T.);
#74082=ORIENTED_EDGE('',*,*,#52595,.T.);
#74083=ORIENTED_EDGE('',*,*,#52596,.T.);
#74084=ORIENTED_EDGE('',*,*,#52597,.T.);
#74085=ORIENTED_EDGE('',*,*,#52598,.T.);
#74086=ORIENTED_EDGE('',*,*,#52599,.T.);
#74087=ORIENTED_EDGE('',*,*,#52600,.T.);
#74088=ORIENTED_EDGE('',*,*,#52601,.T.);
#74089=ORIENTED_EDGE('',*,*,#52602,.T.);
#74090=ORIENTED_EDGE('',*,*,#52603,.T.);
#74091=ORIENTED_EDGE('',*,*,#52050,.T.);
#74092=ORIENTED_EDGE('',*,*,#52603,.F.);
#74093=ORIENTED_EDGE('',*,*,#52604,.T.);
#74094=ORIENTED_EDGE('',*,*,#52605,.T.);
#74095=ORIENTED_EDGE('',*,*,#52606,.T.);
#74096=ORIENTED_EDGE('',*,*,#52607,.T.);
#74097=ORIENTED_EDGE('',*,*,#52608,.T.);
#74098=ORIENTED_EDGE('',*,*,#52609,.T.);
#74099=ORIENTED_EDGE('',*,*,#52610,.T.);
#74100=ORIENTED_EDGE('',*,*,#52611,.T.);
#74101=ORIENTED_EDGE('',*,*,#52612,.T.);
#74102=ORIENTED_EDGE('',*,*,#52613,.T.);
#74103=ORIENTED_EDGE('',*,*,#52614,.T.);
#74104=ORIENTED_EDGE('',*,*,#52615,.T.);
#74105=ORIENTED_EDGE('',*,*,#52616,.T.);
#74106=ORIENTED_EDGE('',*,*,#52617,.T.);
#74107=ORIENTED_EDGE('',*,*,#52618,.T.);
#74108=ORIENTED_EDGE('',*,*,#52619,.T.);
#74109=ORIENTED_EDGE('',*,*,#52620,.T.);
#74110=ORIENTED_EDGE('',*,*,#52621,.T.);
#74111=ORIENTED_EDGE('',*,*,#52622,.T.);
#74112=ORIENTED_EDGE('',*,*,#52623,.T.);
#74113=ORIENTED_EDGE('',*,*,#52624,.T.);
#74114=ORIENTED_EDGE('',*,*,#52625,.T.);
#74115=ORIENTED_EDGE('',*,*,#52626,.T.);
#74116=ORIENTED_EDGE('',*,*,#52627,.T.);
#74117=ORIENTED_EDGE('',*,*,#52628,.T.);
#74118=ORIENTED_EDGE('',*,*,#52629,.T.);
#74119=ORIENTED_EDGE('',*,*,#52630,.T.);
#74120=ORIENTED_EDGE('',*,*,#52631,.T.);
#74121=ORIENTED_EDGE('',*,*,#52632,.T.);
#74122=ORIENTED_EDGE('',*,*,#52633,.T.);
#74123=ORIENTED_EDGE('',*,*,#52634,.T.);
#74124=ORIENTED_EDGE('',*,*,#52635,.T.);
#74125=ORIENTED_EDGE('',*,*,#52636,.T.);
#74126=ORIENTED_EDGE('',*,*,#52637,.T.);
#74127=ORIENTED_EDGE('',*,*,#52638,.T.);
#74128=ORIENTED_EDGE('',*,*,#52639,.T.);
#74129=ORIENTED_EDGE('',*,*,#52640,.T.);
#74130=ORIENTED_EDGE('',*,*,#52641,.T.);
#74131=ORIENTED_EDGE('',*,*,#52642,.T.);
#74132=ORIENTED_EDGE('',*,*,#52643,.T.);
#74133=ORIENTED_EDGE('',*,*,#52644,.T.);
#74134=ORIENTED_EDGE('',*,*,#52645,.T.);
#74135=ORIENTED_EDGE('',*,*,#52646,.T.);
#74136=ORIENTED_EDGE('',*,*,#52647,.T.);
#74137=ORIENTED_EDGE('',*,*,#52648,.T.);
#74138=ORIENTED_EDGE('',*,*,#52649,.T.);
#74139=ORIENTED_EDGE('',*,*,#52650,.T.);
#74140=ORIENTED_EDGE('',*,*,#52651,.T.);
#74141=ORIENTED_EDGE('',*,*,#52652,.T.);
#74142=ORIENTED_EDGE('',*,*,#52653,.T.);
#74143=ORIENTED_EDGE('',*,*,#52654,.T.);
#74144=ORIENTED_EDGE('',*,*,#52655,.T.);
#74145=ORIENTED_EDGE('',*,*,#52656,.T.);
#74146=ORIENTED_EDGE('',*,*,#52657,.T.);
#74147=ORIENTED_EDGE('',*,*,#52658,.T.);
#74148=ORIENTED_EDGE('',*,*,#52659,.T.);
#74149=ORIENTED_EDGE('',*,*,#52660,.T.);
#74150=ORIENTED_EDGE('',*,*,#52661,.T.);
#74151=ORIENTED_EDGE('',*,*,#52662,.T.);
#74152=ORIENTED_EDGE('',*,*,#52663,.T.);
#74153=ORIENTED_EDGE('',*,*,#52664,.T.);
#74154=ORIENTED_EDGE('',*,*,#52665,.T.);
#74155=ORIENTED_EDGE('',*,*,#52666,.T.);
#74156=ORIENTED_EDGE('',*,*,#52667,.T.);
#74157=ORIENTED_EDGE('',*,*,#52668,.T.);
#74158=ORIENTED_EDGE('',*,*,#52669,.T.);
#74159=ORIENTED_EDGE('',*,*,#52670,.T.);
#74160=ORIENTED_EDGE('',*,*,#52671,.T.);
#74161=ORIENTED_EDGE('',*,*,#52672,.T.);
#74162=ORIENTED_EDGE('',*,*,#52673,.T.);
#74163=ORIENTED_EDGE('',*,*,#52674,.T.);
#74164=ORIENTED_EDGE('',*,*,#52675,.T.);
#74165=ORIENTED_EDGE('',*,*,#52676,.T.);
#74166=ORIENTED_EDGE('',*,*,#52677,.T.);
#74167=ORIENTED_EDGE('',*,*,#52678,.T.);
#74168=ORIENTED_EDGE('',*,*,#52679,.T.);
#74169=ORIENTED_EDGE('',*,*,#52680,.T.);
#74170=ORIENTED_EDGE('',*,*,#52681,.T.);
#74171=ORIENTED_EDGE('',*,*,#52682,.T.);
#74172=ORIENTED_EDGE('',*,*,#52683,.T.);
#74173=ORIENTED_EDGE('',*,*,#52684,.T.);
#74174=ORIENTED_EDGE('',*,*,#52685,.T.);
#74175=ORIENTED_EDGE('',*,*,#52686,.T.);
#74176=ORIENTED_EDGE('',*,*,#52687,.T.);
#74177=ORIENTED_EDGE('',*,*,#52688,.T.);
#74178=ORIENTED_EDGE('',*,*,#52689,.T.);
#74179=ORIENTED_EDGE('',*,*,#52690,.T.);
#74180=ORIENTED_EDGE('',*,*,#52691,.T.);
#74181=ORIENTED_EDGE('',*,*,#52692,.T.);
#74182=ORIENTED_EDGE('',*,*,#52693,.T.);
#74183=ORIENTED_EDGE('',*,*,#52031,.T.);
#74184=ORIENTED_EDGE('',*,*,#52694,.T.);
#74185=ORIENTED_EDGE('',*,*,#52695,.T.);
#74186=ORIENTED_EDGE('',*,*,#52696,.T.);
#74187=ORIENTED_EDGE('',*,*,#52697,.T.);
#74188=ORIENTED_EDGE('',*,*,#52698,.T.);
#74189=ORIENTED_EDGE('',*,*,#52699,.T.);
#74190=ORIENTED_EDGE('',*,*,#52700,.T.);
#74191=ORIENTED_EDGE('',*,*,#52701,.T.);
#74192=ORIENTED_EDGE('',*,*,#52702,.T.);
#74193=ORIENTED_EDGE('',*,*,#52703,.T.);
#74194=ORIENTED_EDGE('',*,*,#52704,.T.);
#74195=ORIENTED_EDGE('',*,*,#52705,.T.);
#74196=ORIENTED_EDGE('',*,*,#52706,.T.);
#74197=ORIENTED_EDGE('',*,*,#52707,.T.);
#74198=ORIENTED_EDGE('',*,*,#52708,.T.);
#74199=ORIENTED_EDGE('',*,*,#52709,.T.);
#74200=ORIENTED_EDGE('',*,*,#52710,.T.);
#74201=ORIENTED_EDGE('',*,*,#52711,.T.);
#74202=ORIENTED_EDGE('',*,*,#52712,.T.);
#74203=ORIENTED_EDGE('',*,*,#52713,.T.);
#74204=ORIENTED_EDGE('',*,*,#52714,.T.);
#74205=ORIENTED_EDGE('',*,*,#52715,.T.);
#74206=ORIENTED_EDGE('',*,*,#52716,.T.);
#74207=ORIENTED_EDGE('',*,*,#52717,.T.);
#74208=ORIENTED_EDGE('',*,*,#52718,.T.);
#74209=ORIENTED_EDGE('',*,*,#52719,.T.);
#74210=ORIENTED_EDGE('',*,*,#52720,.T.);
#74211=ORIENTED_EDGE('',*,*,#52721,.T.);
#74212=ORIENTED_EDGE('',*,*,#52722,.T.);
#74213=ORIENTED_EDGE('',*,*,#52723,.T.);
#74214=ORIENTED_EDGE('',*,*,#52724,.T.);
#74215=ORIENTED_EDGE('',*,*,#52725,.T.);
#74216=ORIENTED_EDGE('',*,*,#52726,.T.);
#74217=ORIENTED_EDGE('',*,*,#52727,.T.);
#74218=ORIENTED_EDGE('',*,*,#52728,.T.);
#74219=ORIENTED_EDGE('',*,*,#52729,.T.);
#74220=ORIENTED_EDGE('',*,*,#52730,.T.);
#74221=ORIENTED_EDGE('',*,*,#52731,.T.);
#74222=ORIENTED_EDGE('',*,*,#52732,.T.);
#74223=ORIENTED_EDGE('',*,*,#52733,.T.);
#74224=ORIENTED_EDGE('',*,*,#52734,.T.);
#74225=ORIENTED_EDGE('',*,*,#52735,.T.);
#74226=ORIENTED_EDGE('',*,*,#52736,.T.);
#74227=ORIENTED_EDGE('',*,*,#52737,.T.);
#74228=ORIENTED_EDGE('',*,*,#52738,.T.);
#74229=ORIENTED_EDGE('',*,*,#52739,.T.);
#74230=ORIENTED_EDGE('',*,*,#52740,.T.);
#74231=ORIENTED_EDGE('',*,*,#52741,.T.);
#74232=ORIENTED_EDGE('',*,*,#52742,.T.);
#74233=ORIENTED_EDGE('',*,*,#52743,.T.);
#74234=ORIENTED_EDGE('',*,*,#52744,.T.);
#74235=ORIENTED_EDGE('',*,*,#52745,.T.);
#74236=ORIENTED_EDGE('',*,*,#52746,.T.);
#74237=ORIENTED_EDGE('',*,*,#52747,.T.);
#74238=ORIENTED_EDGE('',*,*,#52748,.T.);
#74239=ORIENTED_EDGE('',*,*,#52749,.T.);
#74240=ORIENTED_EDGE('',*,*,#52750,.T.);
#74241=ORIENTED_EDGE('',*,*,#52751,.T.);
#74242=ORIENTED_EDGE('',*,*,#52752,.T.);
#74243=ORIENTED_EDGE('',*,*,#52753,.T.);
#74244=ORIENTED_EDGE('',*,*,#52754,.T.);
#74245=ORIENTED_EDGE('',*,*,#52755,.T.);
#74246=ORIENTED_EDGE('',*,*,#52756,.T.);
#74247=ORIENTED_EDGE('',*,*,#52757,.T.);
#74248=ORIENTED_EDGE('',*,*,#52758,.T.);
#74249=ORIENTED_EDGE('',*,*,#52759,.T.);
#74250=ORIENTED_EDGE('',*,*,#52760,.T.);
#74251=ORIENTED_EDGE('',*,*,#52761,.T.);
#74252=ORIENTED_EDGE('',*,*,#52762,.T.);
#74253=ORIENTED_EDGE('',*,*,#52763,.T.);
#74254=ORIENTED_EDGE('',*,*,#52764,.T.);
#74255=ORIENTED_EDGE('',*,*,#52765,.T.);
#74256=ORIENTED_EDGE('',*,*,#52766,.T.);
#74257=ORIENTED_EDGE('',*,*,#52767,.T.);
#74258=ORIENTED_EDGE('',*,*,#52768,.T.);
#74259=ORIENTED_EDGE('',*,*,#52769,.T.);
#74260=ORIENTED_EDGE('',*,*,#52770,.T.);
#74261=ORIENTED_EDGE('',*,*,#52771,.T.);
#74262=ORIENTED_EDGE('',*,*,#52772,.T.);
#74263=ORIENTED_EDGE('',*,*,#52773,.T.);
#74264=ORIENTED_EDGE('',*,*,#52774,.T.);
#74265=ORIENTED_EDGE('',*,*,#52775,.T.);
#74266=ORIENTED_EDGE('',*,*,#52776,.T.);
#74267=ORIENTED_EDGE('',*,*,#52777,.T.);
#74268=ORIENTED_EDGE('',*,*,#52778,.T.);
#74269=ORIENTED_EDGE('',*,*,#52779,.T.);
#74270=ORIENTED_EDGE('',*,*,#52780,.T.);
#74271=ORIENTED_EDGE('',*,*,#52781,.T.);
#74272=ORIENTED_EDGE('',*,*,#52782,.T.);
#74273=ORIENTED_EDGE('',*,*,#52783,.T.);
#74274=ORIENTED_EDGE('',*,*,#52784,.T.);
#74275=ORIENTED_EDGE('',*,*,#52048,.T.);
#74276=ORIENTED_EDGE('',*,*,#52049,.T.);
#74277=ORIENTED_EDGE('',*,*,#52784,.F.);
#74278=ORIENTED_EDGE('',*,*,#52785,.T.);
#74279=ORIENTED_EDGE('',*,*,#52783,.F.);
#74280=ORIENTED_EDGE('',*,*,#52786,.T.);
#74281=ORIENTED_EDGE('',*,*,#52787,.T.);
#74282=ORIENTED_EDGE('',*,*,#52786,.F.);
#74283=ORIENTED_EDGE('',*,*,#52785,.F.);
#74284=ORIENTED_EDGE('',*,*,#52788,.F.);
#74285=ORIENTED_EDGE('',*,*,#52789,.T.);
#74286=ORIENTED_EDGE('',*,*,#52790,.T.);
#74287=ORIENTED_EDGE('',*,*,#52791,.T.);
#74288=ORIENTED_EDGE('',*,*,#52792,.F.);
#74289=ORIENTED_EDGE('',*,*,#52793,.F.);
#74290=ORIENTED_EDGE('',*,*,#52794,.T.);
#74291=ORIENTED_EDGE('',*,*,#52795,.T.);
#74292=ORIENTED_EDGE('',*,*,#52793,.T.);
#74293=ORIENTED_EDGE('',*,*,#52796,.T.);
#74294=ORIENTED_EDGE('',*,*,#52797,.T.);
#74295=ORIENTED_EDGE('',*,*,#52798,.T.);
#74296=ORIENTED_EDGE('',*,*,#52799,.T.);
#74297=ORIENTED_EDGE('',*,*,#52800,.T.);
#74298=ORIENTED_EDGE('',*,*,#52801,.F.);
#74299=ORIENTED_EDGE('',*,*,#52802,.T.);
#74300=ORIENTED_EDGE('',*,*,#52803,.T.);
#74301=ORIENTED_EDGE('',*,*,#52804,.T.);
#74302=ORIENTED_EDGE('',*,*,#52805,.F.);
#74303=ORIENTED_EDGE('',*,*,#52806,.F.);
#74304=ORIENTED_EDGE('',*,*,#52807,.T.);
#74305=ORIENTED_EDGE('',*,*,#52808,.T.);
#74306=ORIENTED_EDGE('',*,*,#52806,.T.);
#74307=ORIENTED_EDGE('',*,*,#52809,.T.);
#74308=ORIENTED_EDGE('',*,*,#52790,.F.);
#74309=ORIENTED_EDGE('',*,*,#52810,.T.);
#74310=ORIENTED_EDGE('',*,*,#52607,.F.);
#74311=ORIENTED_EDGE('',*,*,#52811,.T.);
#74312=ORIENTED_EDGE('',*,*,#52420,.F.);
#74313=ORIENTED_EDGE('',*,*,#52812,.T.);
#74314=ORIENTED_EDGE('',*,*,#52807,.F.);
#74315=ORIENTED_EDGE('',*,*,#52813,.T.);
#74316=ORIENTED_EDGE('',*,*,#52803,.F.);
#74317=ORIENTED_EDGE('',*,*,#52814,.T.);
#74318=ORIENTED_EDGE('',*,*,#52797,.F.);
#74319=ORIENTED_EDGE('',*,*,#52815,.T.);
#74320=ORIENTED_EDGE('',*,*,#52799,.F.);
#74321=ORIENTED_EDGE('',*,*,#52816,.T.);
#74322=ORIENTED_EDGE('',*,*,#52794,.F.);
#74323=ORIENTED_EDGE('',*,*,#52817,.T.);
#74324=ORIENTED_EDGE('',*,*,#52818,.T.);
#74325=ORIENTED_EDGE('',*,*,#52819,.T.);
#74326=ORIENTED_EDGE('',*,*,#52820,.F.);
#74327=ORIENTED_EDGE('',*,*,#52821,.F.);
#74328=ORIENTED_EDGE('',*,*,#52822,.F.);
#74329=ORIENTED_EDGE('',*,*,#52823,.T.);
#74330=ORIENTED_EDGE('',*,*,#52821,.T.);
#74331=ORIENTED_EDGE('',*,*,#52824,.T.);
#74332=ORIENTED_EDGE('',*,*,#52825,.T.);
#74333=ORIENTED_EDGE('',*,*,#52826,.T.);
#74334=ORIENTED_EDGE('',*,*,#52827,.T.);
#74335=ORIENTED_EDGE('',*,*,#52828,.T.);
#74336=ORIENTED_EDGE('',*,*,#52829,.T.);
#74337=ORIENTED_EDGE('',*,*,#52830,.T.);
#74338=ORIENTED_EDGE('',*,*,#52831,.T.);
#74339=ORIENTED_EDGE('',*,*,#52832,.T.);
#74340=ORIENTED_EDGE('',*,*,#52833,.F.);
#74341=ORIENTED_EDGE('',*,*,#52834,.F.);
#74342=ORIENTED_EDGE('',*,*,#52835,.F.);
#74343=ORIENTED_EDGE('',*,*,#52836,.T.);
#74344=ORIENTED_EDGE('',*,*,#52834,.T.);
#74345=ORIENTED_EDGE('',*,*,#52837,.T.);
#74346=ORIENTED_EDGE('',*,*,#52838,.T.);
#74347=ORIENTED_EDGE('',*,*,#52839,.T.);
#74348=ORIENTED_EDGE('',*,*,#52613,.F.);
#74349=ORIENTED_EDGE('',*,*,#52840,.T.);
#74350=ORIENTED_EDGE('',*,*,#52818,.F.);
#74351=ORIENTED_EDGE('',*,*,#52841,.T.);
#74352=ORIENTED_EDGE('',*,*,#52838,.F.);
#74353=ORIENTED_EDGE('',*,*,#52842,.T.);
#74354=ORIENTED_EDGE('',*,*,#52414,.F.);
#74355=ORIENTED_EDGE('',*,*,#52843,.T.);
#74356=ORIENTED_EDGE('',*,*,#52829,.F.);
#74357=ORIENTED_EDGE('',*,*,#52844,.T.);
#74358=ORIENTED_EDGE('',*,*,#52831,.F.);
#74359=ORIENTED_EDGE('',*,*,#52845,.T.);
#74360=ORIENTED_EDGE('',*,*,#52825,.F.);
#74361=ORIENTED_EDGE('',*,*,#52846,.T.);
#74362=ORIENTED_EDGE('',*,*,#52827,.F.);
#74363=ORIENTED_EDGE('',*,*,#52847,.T.);
#74364=ORIENTED_EDGE('',*,*,#52848,.T.);
#74365=ORIENTED_EDGE('',*,*,#52849,.T.);
#74366=ORIENTED_EDGE('',*,*,#52850,.F.);
#74367=ORIENTED_EDGE('',*,*,#52851,.F.);
#74368=ORIENTED_EDGE('',*,*,#52852,.F.);
#74369=ORIENTED_EDGE('',*,*,#52853,.T.);
#74370=ORIENTED_EDGE('',*,*,#52851,.T.);
#74371=ORIENTED_EDGE('',*,*,#52854,.T.);
#74372=ORIENTED_EDGE('',*,*,#52855,.T.);
#74373=ORIENTED_EDGE('',*,*,#52856,.T.);
#74374=ORIENTED_EDGE('',*,*,#52857,.T.);
#74375=ORIENTED_EDGE('',*,*,#52858,.T.);
#74376=ORIENTED_EDGE('',*,*,#52859,.T.);
#74377=ORIENTED_EDGE('',*,*,#52860,.T.);
#74378=ORIENTED_EDGE('',*,*,#52861,.T.);
#74379=ORIENTED_EDGE('',*,*,#52862,.T.);
#74380=ORIENTED_EDGE('',*,*,#52863,.F.);
#74381=ORIENTED_EDGE('',*,*,#52864,.F.);
#74382=ORIENTED_EDGE('',*,*,#52865,.F.);
#74383=ORIENTED_EDGE('',*,*,#52866,.T.);
#74384=ORIENTED_EDGE('',*,*,#52864,.T.);
#74385=ORIENTED_EDGE('',*,*,#52867,.T.);
#74386=ORIENTED_EDGE('',*,*,#52868,.T.);
#74387=ORIENTED_EDGE('',*,*,#52869,.T.);
#74388=ORIENTED_EDGE('',*,*,#52619,.F.);
#74389=ORIENTED_EDGE('',*,*,#52870,.T.);
#74390=ORIENTED_EDGE('',*,*,#52848,.F.);
#74391=ORIENTED_EDGE('',*,*,#52871,.T.);
#74392=ORIENTED_EDGE('',*,*,#52868,.F.);
#74393=ORIENTED_EDGE('',*,*,#52872,.T.);
#74394=ORIENTED_EDGE('',*,*,#52408,.F.);
#74395=ORIENTED_EDGE('',*,*,#52873,.T.);
#74396=ORIENTED_EDGE('',*,*,#52859,.F.);
#74397=ORIENTED_EDGE('',*,*,#52874,.T.);
#74398=ORIENTED_EDGE('',*,*,#52861,.F.);
#74399=ORIENTED_EDGE('',*,*,#52875,.T.);
#74400=ORIENTED_EDGE('',*,*,#52855,.F.);
#74401=ORIENTED_EDGE('',*,*,#52876,.T.);
#74402=ORIENTED_EDGE('',*,*,#52857,.F.);
#74403=ORIENTED_EDGE('',*,*,#52877,.T.);
#74404=ORIENTED_EDGE('',*,*,#52878,.T.);
#74405=ORIENTED_EDGE('',*,*,#52879,.T.);
#74406=ORIENTED_EDGE('',*,*,#52880,.F.);
#74407=ORIENTED_EDGE('',*,*,#52881,.F.);
#74408=ORIENTED_EDGE('',*,*,#52882,.F.);
#74409=ORIENTED_EDGE('',*,*,#52883,.T.);
#74410=ORIENTED_EDGE('',*,*,#52881,.T.);
#74411=ORIENTED_EDGE('',*,*,#52884,.T.);
#74412=ORIENTED_EDGE('',*,*,#52885,.T.);
#74413=ORIENTED_EDGE('',*,*,#52886,.T.);
#74414=ORIENTED_EDGE('',*,*,#52887,.T.);
#74415=ORIENTED_EDGE('',*,*,#52888,.T.);
#74416=ORIENTED_EDGE('',*,*,#52889,.T.);
#74417=ORIENTED_EDGE('',*,*,#52890,.T.);
#74418=ORIENTED_EDGE('',*,*,#52891,.T.);
#74419=ORIENTED_EDGE('',*,*,#52892,.T.);
#74420=ORIENTED_EDGE('',*,*,#52893,.F.);
#74421=ORIENTED_EDGE('',*,*,#52894,.F.);
#74422=ORIENTED_EDGE('',*,*,#52895,.F.);
#74423=ORIENTED_EDGE('',*,*,#52896,.T.);
#74424=ORIENTED_EDGE('',*,*,#52894,.T.);
#74425=ORIENTED_EDGE('',*,*,#52897,.T.);
#74426=ORIENTED_EDGE('',*,*,#52898,.T.);
#74427=ORIENTED_EDGE('',*,*,#52899,.T.);
#74428=ORIENTED_EDGE('',*,*,#52625,.F.);
#74429=ORIENTED_EDGE('',*,*,#52900,.T.);
#74430=ORIENTED_EDGE('',*,*,#52878,.F.);
#74431=ORIENTED_EDGE('',*,*,#52901,.T.);
#74432=ORIENTED_EDGE('',*,*,#52898,.F.);
#74433=ORIENTED_EDGE('',*,*,#52902,.T.);
#74434=ORIENTED_EDGE('',*,*,#52402,.F.);
#74435=ORIENTED_EDGE('',*,*,#52903,.T.);
#74436=ORIENTED_EDGE('',*,*,#52889,.F.);
#74437=ORIENTED_EDGE('',*,*,#52904,.T.);
#74438=ORIENTED_EDGE('',*,*,#52891,.F.);
#74439=ORIENTED_EDGE('',*,*,#52905,.T.);
#74440=ORIENTED_EDGE('',*,*,#52885,.F.);
#74441=ORIENTED_EDGE('',*,*,#52906,.T.);
#74442=ORIENTED_EDGE('',*,*,#52887,.F.);
#74443=ORIENTED_EDGE('',*,*,#52907,.T.);
#74444=ORIENTED_EDGE('',*,*,#52908,.T.);
#74445=ORIENTED_EDGE('',*,*,#52909,.T.);
#74446=ORIENTED_EDGE('',*,*,#52910,.F.);
#74447=ORIENTED_EDGE('',*,*,#52911,.F.);
#74448=ORIENTED_EDGE('',*,*,#52912,.F.);
#74449=ORIENTED_EDGE('',*,*,#52913,.T.);
#74450=ORIENTED_EDGE('',*,*,#52911,.T.);
#74451=ORIENTED_EDGE('',*,*,#52914,.T.);
#74452=ORIENTED_EDGE('',*,*,#52915,.T.);
#74453=ORIENTED_EDGE('',*,*,#52916,.T.);
#74454=ORIENTED_EDGE('',*,*,#52917,.T.);
#74455=ORIENTED_EDGE('',*,*,#52918,.T.);
#74456=ORIENTED_EDGE('',*,*,#52919,.T.);
#74457=ORIENTED_EDGE('',*,*,#52920,.T.);
#74458=ORIENTED_EDGE('',*,*,#52921,.T.);
#74459=ORIENTED_EDGE('',*,*,#52922,.T.);
#74460=ORIENTED_EDGE('',*,*,#52923,.F.);
#74461=ORIENTED_EDGE('',*,*,#52924,.F.);
#74462=ORIENTED_EDGE('',*,*,#52925,.F.);
#74463=ORIENTED_EDGE('',*,*,#52926,.T.);
#74464=ORIENTED_EDGE('',*,*,#52924,.T.);
#74465=ORIENTED_EDGE('',*,*,#52927,.T.);
#74466=ORIENTED_EDGE('',*,*,#52928,.T.);
#74467=ORIENTED_EDGE('',*,*,#52929,.T.);
#74468=ORIENTED_EDGE('',*,*,#52631,.F.);
#74469=ORIENTED_EDGE('',*,*,#52930,.T.);
#74470=ORIENTED_EDGE('',*,*,#52908,.F.);
#74471=ORIENTED_EDGE('',*,*,#52931,.T.);
#74472=ORIENTED_EDGE('',*,*,#52928,.F.);
#74473=ORIENTED_EDGE('',*,*,#52932,.T.);
#74474=ORIENTED_EDGE('',*,*,#52396,.F.);
#74475=ORIENTED_EDGE('',*,*,#52933,.T.);
#74476=ORIENTED_EDGE('',*,*,#52919,.F.);
#74477=ORIENTED_EDGE('',*,*,#52934,.T.);
#74478=ORIENTED_EDGE('',*,*,#52921,.F.);
#74479=ORIENTED_EDGE('',*,*,#52935,.T.);
#74480=ORIENTED_EDGE('',*,*,#52915,.F.);
#74481=ORIENTED_EDGE('',*,*,#52936,.T.);
#74482=ORIENTED_EDGE('',*,*,#52917,.F.);
#74483=ORIENTED_EDGE('',*,*,#52937,.T.);
#74484=ORIENTED_EDGE('',*,*,#52938,.T.);
#74485=ORIENTED_EDGE('',*,*,#52939,.T.);
#74486=ORIENTED_EDGE('',*,*,#52940,.F.);
#74487=ORIENTED_EDGE('',*,*,#52941,.F.);
#74488=ORIENTED_EDGE('',*,*,#52942,.F.);
#74489=ORIENTED_EDGE('',*,*,#52943,.T.);
#74490=ORIENTED_EDGE('',*,*,#52941,.T.);
#74491=ORIENTED_EDGE('',*,*,#52944,.T.);
#74492=ORIENTED_EDGE('',*,*,#52945,.T.);
#74493=ORIENTED_EDGE('',*,*,#52946,.T.);
#74494=ORIENTED_EDGE('',*,*,#52947,.T.);
#74495=ORIENTED_EDGE('',*,*,#52948,.T.);
#74496=ORIENTED_EDGE('',*,*,#52949,.T.);
#74497=ORIENTED_EDGE('',*,*,#52950,.T.);
#74498=ORIENTED_EDGE('',*,*,#52951,.T.);
#74499=ORIENTED_EDGE('',*,*,#52952,.T.);
#74500=ORIENTED_EDGE('',*,*,#52953,.F.);
#74501=ORIENTED_EDGE('',*,*,#52954,.F.);
#74502=ORIENTED_EDGE('',*,*,#52955,.F.);
#74503=ORIENTED_EDGE('',*,*,#52956,.T.);
#74504=ORIENTED_EDGE('',*,*,#52954,.T.);
#74505=ORIENTED_EDGE('',*,*,#52957,.T.);
#74506=ORIENTED_EDGE('',*,*,#52958,.T.);
#74507=ORIENTED_EDGE('',*,*,#52959,.T.);
#74508=ORIENTED_EDGE('',*,*,#52637,.F.);
#74509=ORIENTED_EDGE('',*,*,#52960,.T.);
#74510=ORIENTED_EDGE('',*,*,#52938,.F.);
#74511=ORIENTED_EDGE('',*,*,#52961,.T.);
#74512=ORIENTED_EDGE('',*,*,#52958,.F.);
#74513=ORIENTED_EDGE('',*,*,#52962,.T.);
#74514=ORIENTED_EDGE('',*,*,#52390,.F.);
#74515=ORIENTED_EDGE('',*,*,#52963,.T.);
#74516=ORIENTED_EDGE('',*,*,#52949,.F.);
#74517=ORIENTED_EDGE('',*,*,#52964,.T.);
#74518=ORIENTED_EDGE('',*,*,#52951,.F.);
#74519=ORIENTED_EDGE('',*,*,#52965,.T.);
#74520=ORIENTED_EDGE('',*,*,#52945,.F.);
#74521=ORIENTED_EDGE('',*,*,#52966,.T.);
#74522=ORIENTED_EDGE('',*,*,#52947,.F.);
#74523=ORIENTED_EDGE('',*,*,#52967,.T.);
#74524=ORIENTED_EDGE('',*,*,#52968,.T.);
#74525=ORIENTED_EDGE('',*,*,#52969,.T.);
#74526=ORIENTED_EDGE('',*,*,#52970,.F.);
#74527=ORIENTED_EDGE('',*,*,#52971,.F.);
#74528=ORIENTED_EDGE('',*,*,#52972,.F.);
#74529=ORIENTED_EDGE('',*,*,#52973,.T.);
#74530=ORIENTED_EDGE('',*,*,#52971,.T.);
#74531=ORIENTED_EDGE('',*,*,#52974,.T.);
#74532=ORIENTED_EDGE('',*,*,#52975,.T.);
#74533=ORIENTED_EDGE('',*,*,#52976,.T.);
#74534=ORIENTED_EDGE('',*,*,#52977,.T.);
#74535=ORIENTED_EDGE('',*,*,#52978,.T.);
#74536=ORIENTED_EDGE('',*,*,#52979,.T.);
#74537=ORIENTED_EDGE('',*,*,#52980,.T.);
#74538=ORIENTED_EDGE('',*,*,#52981,.T.);
#74539=ORIENTED_EDGE('',*,*,#52982,.T.);
#74540=ORIENTED_EDGE('',*,*,#52983,.F.);
#74541=ORIENTED_EDGE('',*,*,#52984,.F.);
#74542=ORIENTED_EDGE('',*,*,#52985,.F.);
#74543=ORIENTED_EDGE('',*,*,#52986,.T.);
#74544=ORIENTED_EDGE('',*,*,#52984,.T.);
#74545=ORIENTED_EDGE('',*,*,#52987,.T.);
#74546=ORIENTED_EDGE('',*,*,#52988,.T.);
#74547=ORIENTED_EDGE('',*,*,#52989,.T.);
#74548=ORIENTED_EDGE('',*,*,#52643,.F.);
#74549=ORIENTED_EDGE('',*,*,#52990,.T.);
#74550=ORIENTED_EDGE('',*,*,#52968,.F.);
#74551=ORIENTED_EDGE('',*,*,#52991,.T.);
#74552=ORIENTED_EDGE('',*,*,#52988,.F.);
#74553=ORIENTED_EDGE('',*,*,#52992,.T.);
#74554=ORIENTED_EDGE('',*,*,#52384,.F.);
#74555=ORIENTED_EDGE('',*,*,#52993,.T.);
#74556=ORIENTED_EDGE('',*,*,#52979,.F.);
#74557=ORIENTED_EDGE('',*,*,#52994,.T.);
#74558=ORIENTED_EDGE('',*,*,#52981,.F.);
#74559=ORIENTED_EDGE('',*,*,#52995,.T.);
#74560=ORIENTED_EDGE('',*,*,#52975,.F.);
#74561=ORIENTED_EDGE('',*,*,#52996,.T.);
#74562=ORIENTED_EDGE('',*,*,#52977,.F.);
#74563=ORIENTED_EDGE('',*,*,#52997,.T.);
#74564=ORIENTED_EDGE('',*,*,#52998,.T.);
#74565=ORIENTED_EDGE('',*,*,#52999,.T.);
#74566=ORIENTED_EDGE('',*,*,#53000,.F.);
#74567=ORIENTED_EDGE('',*,*,#53001,.F.);
#74568=ORIENTED_EDGE('',*,*,#53002,.F.);
#74569=ORIENTED_EDGE('',*,*,#53003,.T.);
#74570=ORIENTED_EDGE('',*,*,#53001,.T.);
#74571=ORIENTED_EDGE('',*,*,#53004,.T.);
#74572=ORIENTED_EDGE('',*,*,#53005,.T.);
#74573=ORIENTED_EDGE('',*,*,#53006,.T.);
#74574=ORIENTED_EDGE('',*,*,#53007,.T.);
#74575=ORIENTED_EDGE('',*,*,#53008,.T.);
#74576=ORIENTED_EDGE('',*,*,#53009,.T.);
#74577=ORIENTED_EDGE('',*,*,#53010,.T.);
#74578=ORIENTED_EDGE('',*,*,#53011,.T.);
#74579=ORIENTED_EDGE('',*,*,#53012,.T.);
#74580=ORIENTED_EDGE('',*,*,#53013,.F.);
#74581=ORIENTED_EDGE('',*,*,#53014,.F.);
#74582=ORIENTED_EDGE('',*,*,#53015,.F.);
#74583=ORIENTED_EDGE('',*,*,#53016,.T.);
#74584=ORIENTED_EDGE('',*,*,#53014,.T.);
#74585=ORIENTED_EDGE('',*,*,#53017,.T.);
#74586=ORIENTED_EDGE('',*,*,#53018,.T.);
#74587=ORIENTED_EDGE('',*,*,#53019,.T.);
#74588=ORIENTED_EDGE('',*,*,#52649,.F.);
#74589=ORIENTED_EDGE('',*,*,#53020,.T.);
#74590=ORIENTED_EDGE('',*,*,#52998,.F.);
#74591=ORIENTED_EDGE('',*,*,#53021,.T.);
#74592=ORIENTED_EDGE('',*,*,#53018,.F.);
#74593=ORIENTED_EDGE('',*,*,#53022,.T.);
#74594=ORIENTED_EDGE('',*,*,#52378,.F.);
#74595=ORIENTED_EDGE('',*,*,#53023,.T.);
#74596=ORIENTED_EDGE('',*,*,#53009,.F.);
#74597=ORIENTED_EDGE('',*,*,#53024,.T.);
#74598=ORIENTED_EDGE('',*,*,#53011,.F.);
#74599=ORIENTED_EDGE('',*,*,#53025,.T.);
#74600=ORIENTED_EDGE('',*,*,#53005,.F.);
#74601=ORIENTED_EDGE('',*,*,#53026,.T.);
#74602=ORIENTED_EDGE('',*,*,#53007,.F.);
#74603=ORIENTED_EDGE('',*,*,#53027,.T.);
#74604=ORIENTED_EDGE('',*,*,#53028,.T.);
#74605=ORIENTED_EDGE('',*,*,#53029,.T.);
#74606=ORIENTED_EDGE('',*,*,#53030,.F.);
#74607=ORIENTED_EDGE('',*,*,#53031,.F.);
#74608=ORIENTED_EDGE('',*,*,#53032,.F.);
#74609=ORIENTED_EDGE('',*,*,#53033,.T.);
#74610=ORIENTED_EDGE('',*,*,#53031,.T.);
#74611=ORIENTED_EDGE('',*,*,#53034,.T.);
#74612=ORIENTED_EDGE('',*,*,#53035,.T.);
#74613=ORIENTED_EDGE('',*,*,#53036,.T.);
#74614=ORIENTED_EDGE('',*,*,#53037,.T.);
#74615=ORIENTED_EDGE('',*,*,#53038,.T.);
#74616=ORIENTED_EDGE('',*,*,#53039,.T.);
#74617=ORIENTED_EDGE('',*,*,#53040,.T.);
#74618=ORIENTED_EDGE('',*,*,#53041,.T.);
#74619=ORIENTED_EDGE('',*,*,#53042,.T.);
#74620=ORIENTED_EDGE('',*,*,#53043,.F.);
#74621=ORIENTED_EDGE('',*,*,#53044,.F.);
#74622=ORIENTED_EDGE('',*,*,#53045,.F.);
#74623=ORIENTED_EDGE('',*,*,#53046,.T.);
#74624=ORIENTED_EDGE('',*,*,#53044,.T.);
#74625=ORIENTED_EDGE('',*,*,#53047,.T.);
#74626=ORIENTED_EDGE('',*,*,#53048,.T.);
#74627=ORIENTED_EDGE('',*,*,#53049,.T.);
#74628=ORIENTED_EDGE('',*,*,#52655,.F.);
#74629=ORIENTED_EDGE('',*,*,#53050,.T.);
#74630=ORIENTED_EDGE('',*,*,#53028,.F.);
#74631=ORIENTED_EDGE('',*,*,#53051,.T.);
#74632=ORIENTED_EDGE('',*,*,#53048,.F.);
#74633=ORIENTED_EDGE('',*,*,#53052,.T.);
#74634=ORIENTED_EDGE('',*,*,#52372,.F.);
#74635=ORIENTED_EDGE('',*,*,#53053,.T.);
#74636=ORIENTED_EDGE('',*,*,#53039,.F.);
#74637=ORIENTED_EDGE('',*,*,#53054,.T.);
#74638=ORIENTED_EDGE('',*,*,#53041,.F.);
#74639=ORIENTED_EDGE('',*,*,#53055,.T.);
#74640=ORIENTED_EDGE('',*,*,#53035,.F.);
#74641=ORIENTED_EDGE('',*,*,#53056,.T.);
#74642=ORIENTED_EDGE('',*,*,#53037,.F.);
#74643=ORIENTED_EDGE('',*,*,#53057,.T.);
#74644=ORIENTED_EDGE('',*,*,#53058,.T.);
#74645=ORIENTED_EDGE('',*,*,#53059,.T.);
#74646=ORIENTED_EDGE('',*,*,#53060,.F.);
#74647=ORIENTED_EDGE('',*,*,#53061,.F.);
#74648=ORIENTED_EDGE('',*,*,#53062,.F.);
#74649=ORIENTED_EDGE('',*,*,#53063,.T.);
#74650=ORIENTED_EDGE('',*,*,#53061,.T.);
#74651=ORIENTED_EDGE('',*,*,#53064,.T.);
#74652=ORIENTED_EDGE('',*,*,#53065,.T.);
#74653=ORIENTED_EDGE('',*,*,#53066,.T.);
#74654=ORIENTED_EDGE('',*,*,#53067,.T.);
#74655=ORIENTED_EDGE('',*,*,#53068,.T.);
#74656=ORIENTED_EDGE('',*,*,#53069,.T.);
#74657=ORIENTED_EDGE('',*,*,#53070,.T.);
#74658=ORIENTED_EDGE('',*,*,#53071,.T.);
#74659=ORIENTED_EDGE('',*,*,#53072,.T.);
#74660=ORIENTED_EDGE('',*,*,#53073,.F.);
#74661=ORIENTED_EDGE('',*,*,#53074,.F.);
#74662=ORIENTED_EDGE('',*,*,#53075,.F.);
#74663=ORIENTED_EDGE('',*,*,#53076,.T.);
#74664=ORIENTED_EDGE('',*,*,#53074,.T.);
#74665=ORIENTED_EDGE('',*,*,#53077,.T.);
#74666=ORIENTED_EDGE('',*,*,#53078,.T.);
#74667=ORIENTED_EDGE('',*,*,#53079,.T.);
#74668=ORIENTED_EDGE('',*,*,#52661,.F.);
#74669=ORIENTED_EDGE('',*,*,#53080,.T.);
#74670=ORIENTED_EDGE('',*,*,#53058,.F.);
#74671=ORIENTED_EDGE('',*,*,#53081,.T.);
#74672=ORIENTED_EDGE('',*,*,#53078,.F.);
#74673=ORIENTED_EDGE('',*,*,#53082,.T.);
#74674=ORIENTED_EDGE('',*,*,#52366,.F.);
#74675=ORIENTED_EDGE('',*,*,#53083,.T.);
#74676=ORIENTED_EDGE('',*,*,#53069,.F.);
#74677=ORIENTED_EDGE('',*,*,#53084,.T.);
#74678=ORIENTED_EDGE('',*,*,#53071,.F.);
#74679=ORIENTED_EDGE('',*,*,#53085,.T.);
#74680=ORIENTED_EDGE('',*,*,#53065,.F.);
#74681=ORIENTED_EDGE('',*,*,#53086,.T.);
#74682=ORIENTED_EDGE('',*,*,#53067,.F.);
#74683=ORIENTED_EDGE('',*,*,#53087,.T.);
#74684=ORIENTED_EDGE('',*,*,#53088,.T.);
#74685=ORIENTED_EDGE('',*,*,#53089,.T.);
#74686=ORIENTED_EDGE('',*,*,#53090,.F.);
#74687=ORIENTED_EDGE('',*,*,#53091,.F.);
#74688=ORIENTED_EDGE('',*,*,#53092,.F.);
#74689=ORIENTED_EDGE('',*,*,#53093,.T.);
#74690=ORIENTED_EDGE('',*,*,#53091,.T.);
#74691=ORIENTED_EDGE('',*,*,#53094,.T.);
#74692=ORIENTED_EDGE('',*,*,#53095,.T.);
#74693=ORIENTED_EDGE('',*,*,#53096,.T.);
#74694=ORIENTED_EDGE('',*,*,#53097,.T.);
#74695=ORIENTED_EDGE('',*,*,#53098,.T.);
#74696=ORIENTED_EDGE('',*,*,#53099,.T.);
#74697=ORIENTED_EDGE('',*,*,#53100,.T.);
#74698=ORIENTED_EDGE('',*,*,#53101,.T.);
#74699=ORIENTED_EDGE('',*,*,#53102,.T.);
#74700=ORIENTED_EDGE('',*,*,#53103,.F.);
#74701=ORIENTED_EDGE('',*,*,#53104,.F.);
#74702=ORIENTED_EDGE('',*,*,#53105,.F.);
#74703=ORIENTED_EDGE('',*,*,#53106,.T.);
#74704=ORIENTED_EDGE('',*,*,#53104,.T.);
#74705=ORIENTED_EDGE('',*,*,#53107,.T.);
#74706=ORIENTED_EDGE('',*,*,#53108,.T.);
#74707=ORIENTED_EDGE('',*,*,#53109,.T.);
#74708=ORIENTED_EDGE('',*,*,#52667,.F.);
#74709=ORIENTED_EDGE('',*,*,#53110,.T.);
#74710=ORIENTED_EDGE('',*,*,#53088,.F.);
#74711=ORIENTED_EDGE('',*,*,#53111,.T.);
#74712=ORIENTED_EDGE('',*,*,#53108,.F.);
#74713=ORIENTED_EDGE('',*,*,#53112,.T.);
#74714=ORIENTED_EDGE('',*,*,#52360,.F.);
#74715=ORIENTED_EDGE('',*,*,#53113,.T.);
#74716=ORIENTED_EDGE('',*,*,#53099,.F.);
#74717=ORIENTED_EDGE('',*,*,#53114,.T.);
#74718=ORIENTED_EDGE('',*,*,#53101,.F.);
#74719=ORIENTED_EDGE('',*,*,#53115,.T.);
#74720=ORIENTED_EDGE('',*,*,#53095,.F.);
#74721=ORIENTED_EDGE('',*,*,#53116,.T.);
#74722=ORIENTED_EDGE('',*,*,#53097,.F.);
#74723=ORIENTED_EDGE('',*,*,#53117,.T.);
#74724=ORIENTED_EDGE('',*,*,#53118,.T.);
#74725=ORIENTED_EDGE('',*,*,#53119,.T.);
#74726=ORIENTED_EDGE('',*,*,#53120,.F.);
#74727=ORIENTED_EDGE('',*,*,#53121,.F.);
#74728=ORIENTED_EDGE('',*,*,#53122,.F.);
#74729=ORIENTED_EDGE('',*,*,#53123,.T.);
#74730=ORIENTED_EDGE('',*,*,#53121,.T.);
#74731=ORIENTED_EDGE('',*,*,#53124,.T.);
#74732=ORIENTED_EDGE('',*,*,#53125,.T.);
#74733=ORIENTED_EDGE('',*,*,#53126,.T.);
#74734=ORIENTED_EDGE('',*,*,#53127,.T.);
#74735=ORIENTED_EDGE('',*,*,#53128,.T.);
#74736=ORIENTED_EDGE('',*,*,#53129,.T.);
#74737=ORIENTED_EDGE('',*,*,#53130,.T.);
#74738=ORIENTED_EDGE('',*,*,#53131,.T.);
#74739=ORIENTED_EDGE('',*,*,#53132,.T.);
#74740=ORIENTED_EDGE('',*,*,#53133,.F.);
#74741=ORIENTED_EDGE('',*,*,#53134,.F.);
#74742=ORIENTED_EDGE('',*,*,#53135,.F.);
#74743=ORIENTED_EDGE('',*,*,#53136,.T.);
#74744=ORIENTED_EDGE('',*,*,#53134,.T.);
#74745=ORIENTED_EDGE('',*,*,#53137,.T.);
#74746=ORIENTED_EDGE('',*,*,#53138,.T.);
#74747=ORIENTED_EDGE('',*,*,#53139,.T.);
#74748=ORIENTED_EDGE('',*,*,#52673,.F.);
#74749=ORIENTED_EDGE('',*,*,#53140,.T.);
#74750=ORIENTED_EDGE('',*,*,#53118,.F.);
#74751=ORIENTED_EDGE('',*,*,#53141,.T.);
#74752=ORIENTED_EDGE('',*,*,#53138,.F.);
#74753=ORIENTED_EDGE('',*,*,#53142,.T.);
#74754=ORIENTED_EDGE('',*,*,#52354,.F.);
#74755=ORIENTED_EDGE('',*,*,#53143,.T.);
#74756=ORIENTED_EDGE('',*,*,#53129,.F.);
#74757=ORIENTED_EDGE('',*,*,#53144,.T.);
#74758=ORIENTED_EDGE('',*,*,#53131,.F.);
#74759=ORIENTED_EDGE('',*,*,#53145,.T.);
#74760=ORIENTED_EDGE('',*,*,#53125,.F.);
#74761=ORIENTED_EDGE('',*,*,#53146,.T.);
#74762=ORIENTED_EDGE('',*,*,#53127,.F.);
#74763=ORIENTED_EDGE('',*,*,#53147,.T.);
#74764=ORIENTED_EDGE('',*,*,#53148,.T.);
#74765=ORIENTED_EDGE('',*,*,#53149,.T.);
#74766=ORIENTED_EDGE('',*,*,#53150,.F.);
#74767=ORIENTED_EDGE('',*,*,#53151,.F.);
#74768=ORIENTED_EDGE('',*,*,#53152,.F.);
#74769=ORIENTED_EDGE('',*,*,#53153,.T.);
#74770=ORIENTED_EDGE('',*,*,#53151,.T.);
#74771=ORIENTED_EDGE('',*,*,#53154,.T.);
#74772=ORIENTED_EDGE('',*,*,#53155,.T.);
#74773=ORIENTED_EDGE('',*,*,#53156,.T.);
#74774=ORIENTED_EDGE('',*,*,#53157,.T.);
#74775=ORIENTED_EDGE('',*,*,#53158,.T.);
#74776=ORIENTED_EDGE('',*,*,#53159,.T.);
#74777=ORIENTED_EDGE('',*,*,#53160,.T.);
#74778=ORIENTED_EDGE('',*,*,#53161,.T.);
#74779=ORIENTED_EDGE('',*,*,#53162,.T.);
#74780=ORIENTED_EDGE('',*,*,#53163,.F.);
#74781=ORIENTED_EDGE('',*,*,#53164,.F.);
#74782=ORIENTED_EDGE('',*,*,#53165,.F.);
#74783=ORIENTED_EDGE('',*,*,#53166,.T.);
#74784=ORIENTED_EDGE('',*,*,#53164,.T.);
#74785=ORIENTED_EDGE('',*,*,#53167,.T.);
#74786=ORIENTED_EDGE('',*,*,#53168,.T.);
#74787=ORIENTED_EDGE('',*,*,#53169,.T.);
#74788=ORIENTED_EDGE('',*,*,#52679,.F.);
#74789=ORIENTED_EDGE('',*,*,#53170,.T.);
#74790=ORIENTED_EDGE('',*,*,#53148,.F.);
#74791=ORIENTED_EDGE('',*,*,#53171,.T.);
#74792=ORIENTED_EDGE('',*,*,#53168,.F.);
#74793=ORIENTED_EDGE('',*,*,#53172,.T.);
#74794=ORIENTED_EDGE('',*,*,#52348,.F.);
#74795=ORIENTED_EDGE('',*,*,#53173,.T.);
#74796=ORIENTED_EDGE('',*,*,#53159,.F.);
#74797=ORIENTED_EDGE('',*,*,#53174,.T.);
#74798=ORIENTED_EDGE('',*,*,#53161,.F.);
#74799=ORIENTED_EDGE('',*,*,#53175,.T.);
#74800=ORIENTED_EDGE('',*,*,#53155,.F.);
#74801=ORIENTED_EDGE('',*,*,#53176,.T.);
#74802=ORIENTED_EDGE('',*,*,#53157,.F.);
#74803=ORIENTED_EDGE('',*,*,#53177,.T.);
#74804=ORIENTED_EDGE('',*,*,#53178,.T.);
#74805=ORIENTED_EDGE('',*,*,#53179,.T.);
#74806=ORIENTED_EDGE('',*,*,#53180,.F.);
#74807=ORIENTED_EDGE('',*,*,#53181,.F.);
#74808=ORIENTED_EDGE('',*,*,#53182,.F.);
#74809=ORIENTED_EDGE('',*,*,#53183,.T.);
#74810=ORIENTED_EDGE('',*,*,#53181,.T.);
#74811=ORIENTED_EDGE('',*,*,#53184,.T.);
#74812=ORIENTED_EDGE('',*,*,#53185,.T.);
#74813=ORIENTED_EDGE('',*,*,#53186,.T.);
#74814=ORIENTED_EDGE('',*,*,#53187,.T.);
#74815=ORIENTED_EDGE('',*,*,#53188,.T.);
#74816=ORIENTED_EDGE('',*,*,#53189,.T.);
#74817=ORIENTED_EDGE('',*,*,#53190,.T.);
#74818=ORIENTED_EDGE('',*,*,#53191,.T.);
#74819=ORIENTED_EDGE('',*,*,#53192,.T.);
#74820=ORIENTED_EDGE('',*,*,#53193,.F.);
#74821=ORIENTED_EDGE('',*,*,#53194,.F.);
#74822=ORIENTED_EDGE('',*,*,#53195,.F.);
#74823=ORIENTED_EDGE('',*,*,#53196,.T.);
#74824=ORIENTED_EDGE('',*,*,#53194,.T.);
#74825=ORIENTED_EDGE('',*,*,#53197,.T.);
#74826=ORIENTED_EDGE('',*,*,#53198,.T.);
#74827=ORIENTED_EDGE('',*,*,#53199,.T.);
#74828=ORIENTED_EDGE('',*,*,#52685,.F.);
#74829=ORIENTED_EDGE('',*,*,#53200,.T.);
#74830=ORIENTED_EDGE('',*,*,#53178,.F.);
#74831=ORIENTED_EDGE('',*,*,#53201,.T.);
#74832=ORIENTED_EDGE('',*,*,#53198,.F.);
#74833=ORIENTED_EDGE('',*,*,#53202,.T.);
#74834=ORIENTED_EDGE('',*,*,#52342,.F.);
#74835=ORIENTED_EDGE('',*,*,#53203,.T.);
#74836=ORIENTED_EDGE('',*,*,#53189,.F.);
#74837=ORIENTED_EDGE('',*,*,#53204,.T.);
#74838=ORIENTED_EDGE('',*,*,#53191,.F.);
#74839=ORIENTED_EDGE('',*,*,#53205,.T.);
#74840=ORIENTED_EDGE('',*,*,#53185,.F.);
#74841=ORIENTED_EDGE('',*,*,#53206,.T.);
#74842=ORIENTED_EDGE('',*,*,#53187,.F.);
#74843=ORIENTED_EDGE('',*,*,#53207,.T.);
#74844=ORIENTED_EDGE('',*,*,#53208,.T.);
#74845=ORIENTED_EDGE('',*,*,#53209,.T.);
#74846=ORIENTED_EDGE('',*,*,#53210,.F.);
#74847=ORIENTED_EDGE('',*,*,#53211,.F.);
#74848=ORIENTED_EDGE('',*,*,#53212,.F.);
#74849=ORIENTED_EDGE('',*,*,#53213,.T.);
#74850=ORIENTED_EDGE('',*,*,#53211,.T.);
#74851=ORIENTED_EDGE('',*,*,#53214,.T.);
#74852=ORIENTED_EDGE('',*,*,#53215,.T.);
#74853=ORIENTED_EDGE('',*,*,#53216,.T.);
#74854=ORIENTED_EDGE('',*,*,#53217,.T.);
#74855=ORIENTED_EDGE('',*,*,#53218,.T.);
#74856=ORIENTED_EDGE('',*,*,#53219,.T.);
#74857=ORIENTED_EDGE('',*,*,#53220,.T.);
#74858=ORIENTED_EDGE('',*,*,#53221,.T.);
#74859=ORIENTED_EDGE('',*,*,#53222,.T.);
#74860=ORIENTED_EDGE('',*,*,#53223,.F.);
#74861=ORIENTED_EDGE('',*,*,#53224,.F.);
#74862=ORIENTED_EDGE('',*,*,#53225,.F.);
#74863=ORIENTED_EDGE('',*,*,#53226,.T.);
#74864=ORIENTED_EDGE('',*,*,#53224,.T.);
#74865=ORIENTED_EDGE('',*,*,#53227,.T.);
#74866=ORIENTED_EDGE('',*,*,#53228,.T.);
#74867=ORIENTED_EDGE('',*,*,#53229,.T.);
#74868=ORIENTED_EDGE('',*,*,#52691,.F.);
#74869=ORIENTED_EDGE('',*,*,#53230,.T.);
#74870=ORIENTED_EDGE('',*,*,#53208,.F.);
#74871=ORIENTED_EDGE('',*,*,#53231,.T.);
#74872=ORIENTED_EDGE('',*,*,#53228,.F.);
#74873=ORIENTED_EDGE('',*,*,#53232,.T.);
#74874=ORIENTED_EDGE('',*,*,#52336,.F.);
#74875=ORIENTED_EDGE('',*,*,#53233,.T.);
#74876=ORIENTED_EDGE('',*,*,#53219,.F.);
#74877=ORIENTED_EDGE('',*,*,#53234,.T.);
#74878=ORIENTED_EDGE('',*,*,#53221,.F.);
#74879=ORIENTED_EDGE('',*,*,#53235,.T.);
#74880=ORIENTED_EDGE('',*,*,#53215,.F.);
#74881=ORIENTED_EDGE('',*,*,#53236,.T.);
#74882=ORIENTED_EDGE('',*,*,#53217,.F.);
#74883=ORIENTED_EDGE('',*,*,#53237,.T.);
#74884=ORIENTED_EDGE('',*,*,#53238,.T.);
#74885=ORIENTED_EDGE('',*,*,#53239,.T.);
#74886=ORIENTED_EDGE('',*,*,#53240,.F.);
#74887=ORIENTED_EDGE('',*,*,#53241,.F.);
#74888=ORIENTED_EDGE('',*,*,#53242,.F.);
#74889=ORIENTED_EDGE('',*,*,#53243,.T.);
#74890=ORIENTED_EDGE('',*,*,#53241,.T.);
#74891=ORIENTED_EDGE('',*,*,#53244,.T.);
#74892=ORIENTED_EDGE('',*,*,#53245,.T.);
#74893=ORIENTED_EDGE('',*,*,#53246,.T.);
#74894=ORIENTED_EDGE('',*,*,#53247,.T.);
#74895=ORIENTED_EDGE('',*,*,#53248,.T.);
#74896=ORIENTED_EDGE('',*,*,#53249,.T.);
#74897=ORIENTED_EDGE('',*,*,#53250,.T.);
#74898=ORIENTED_EDGE('',*,*,#53251,.T.);
#74899=ORIENTED_EDGE('',*,*,#53252,.T.);
#74900=ORIENTED_EDGE('',*,*,#53253,.F.);
#74901=ORIENTED_EDGE('',*,*,#53254,.F.);
#74902=ORIENTED_EDGE('',*,*,#53255,.F.);
#74903=ORIENTED_EDGE('',*,*,#53256,.T.);
#74904=ORIENTED_EDGE('',*,*,#53254,.T.);
#74905=ORIENTED_EDGE('',*,*,#53257,.T.);
#74906=ORIENTED_EDGE('',*,*,#53258,.T.);
#74907=ORIENTED_EDGE('',*,*,#53259,.T.);
#74908=ORIENTED_EDGE('',*,*,#52696,.F.);
#74909=ORIENTED_EDGE('',*,*,#53260,.T.);
#74910=ORIENTED_EDGE('',*,*,#53238,.F.);
#74911=ORIENTED_EDGE('',*,*,#53261,.T.);
#74912=ORIENTED_EDGE('',*,*,#53258,.F.);
#74913=ORIENTED_EDGE('',*,*,#53262,.T.);
#74914=ORIENTED_EDGE('',*,*,#52331,.F.);
#74915=ORIENTED_EDGE('',*,*,#53263,.T.);
#74916=ORIENTED_EDGE('',*,*,#53249,.F.);
#74917=ORIENTED_EDGE('',*,*,#53264,.T.);
#74918=ORIENTED_EDGE('',*,*,#53251,.F.);
#74919=ORIENTED_EDGE('',*,*,#53265,.T.);
#74920=ORIENTED_EDGE('',*,*,#53245,.F.);
#74921=ORIENTED_EDGE('',*,*,#53266,.T.);
#74922=ORIENTED_EDGE('',*,*,#53247,.F.);
#74923=ORIENTED_EDGE('',*,*,#53267,.T.);
#74924=ORIENTED_EDGE('',*,*,#53268,.T.);
#74925=ORIENTED_EDGE('',*,*,#53269,.T.);
#74926=ORIENTED_EDGE('',*,*,#53270,.F.);
#74927=ORIENTED_EDGE('',*,*,#53271,.F.);
#74928=ORIENTED_EDGE('',*,*,#53272,.F.);
#74929=ORIENTED_EDGE('',*,*,#53273,.T.);
#74930=ORIENTED_EDGE('',*,*,#53271,.T.);
#74931=ORIENTED_EDGE('',*,*,#53274,.T.);
#74932=ORIENTED_EDGE('',*,*,#53275,.T.);
#74933=ORIENTED_EDGE('',*,*,#53276,.T.);
#74934=ORIENTED_EDGE('',*,*,#53277,.T.);
#74935=ORIENTED_EDGE('',*,*,#53278,.T.);
#74936=ORIENTED_EDGE('',*,*,#53279,.T.);
#74937=ORIENTED_EDGE('',*,*,#53280,.T.);
#74938=ORIENTED_EDGE('',*,*,#53281,.T.);
#74939=ORIENTED_EDGE('',*,*,#53282,.T.);
#74940=ORIENTED_EDGE('',*,*,#53283,.F.);
#74941=ORIENTED_EDGE('',*,*,#53284,.F.);
#74942=ORIENTED_EDGE('',*,*,#53285,.F.);
#74943=ORIENTED_EDGE('',*,*,#53286,.T.);
#74944=ORIENTED_EDGE('',*,*,#53284,.T.);
#74945=ORIENTED_EDGE('',*,*,#53287,.T.);
#74946=ORIENTED_EDGE('',*,*,#53288,.T.);
#74947=ORIENTED_EDGE('',*,*,#53289,.T.);
#74948=ORIENTED_EDGE('',*,*,#52702,.F.);
#74949=ORIENTED_EDGE('',*,*,#53290,.T.);
#74950=ORIENTED_EDGE('',*,*,#53268,.F.);
#74951=ORIENTED_EDGE('',*,*,#53291,.T.);
#74952=ORIENTED_EDGE('',*,*,#53288,.F.);
#74953=ORIENTED_EDGE('',*,*,#53292,.T.);
#74954=ORIENTED_EDGE('',*,*,#52325,.F.);
#74955=ORIENTED_EDGE('',*,*,#53293,.T.);
#74956=ORIENTED_EDGE('',*,*,#53279,.F.);
#74957=ORIENTED_EDGE('',*,*,#53294,.T.);
#74958=ORIENTED_EDGE('',*,*,#53281,.F.);
#74959=ORIENTED_EDGE('',*,*,#53295,.T.);
#74960=ORIENTED_EDGE('',*,*,#53275,.F.);
#74961=ORIENTED_EDGE('',*,*,#53296,.T.);
#74962=ORIENTED_EDGE('',*,*,#53277,.F.);
#74963=ORIENTED_EDGE('',*,*,#53297,.T.);
#74964=ORIENTED_EDGE('',*,*,#53298,.T.);
#74965=ORIENTED_EDGE('',*,*,#53299,.T.);
#74966=ORIENTED_EDGE('',*,*,#53300,.F.);
#74967=ORIENTED_EDGE('',*,*,#53301,.F.);
#74968=ORIENTED_EDGE('',*,*,#53302,.F.);
#74969=ORIENTED_EDGE('',*,*,#53303,.T.);
#74970=ORIENTED_EDGE('',*,*,#53301,.T.);
#74971=ORIENTED_EDGE('',*,*,#53304,.T.);
#74972=ORIENTED_EDGE('',*,*,#53305,.T.);
#74973=ORIENTED_EDGE('',*,*,#53306,.T.);
#74974=ORIENTED_EDGE('',*,*,#53307,.T.);
#74975=ORIENTED_EDGE('',*,*,#53308,.T.);
#74976=ORIENTED_EDGE('',*,*,#53309,.T.);
#74977=ORIENTED_EDGE('',*,*,#53310,.T.);
#74978=ORIENTED_EDGE('',*,*,#53311,.T.);
#74979=ORIENTED_EDGE('',*,*,#53312,.T.);
#74980=ORIENTED_EDGE('',*,*,#53313,.F.);
#74981=ORIENTED_EDGE('',*,*,#53314,.F.);
#74982=ORIENTED_EDGE('',*,*,#53315,.F.);
#74983=ORIENTED_EDGE('',*,*,#53316,.T.);
#74984=ORIENTED_EDGE('',*,*,#53314,.T.);
#74985=ORIENTED_EDGE('',*,*,#53317,.T.);
#74986=ORIENTED_EDGE('',*,*,#53318,.T.);
#74987=ORIENTED_EDGE('',*,*,#53319,.T.);
#74988=ORIENTED_EDGE('',*,*,#52708,.F.);
#74989=ORIENTED_EDGE('',*,*,#53320,.T.);
#74990=ORIENTED_EDGE('',*,*,#53298,.F.);
#74991=ORIENTED_EDGE('',*,*,#53321,.T.);
#74992=ORIENTED_EDGE('',*,*,#53318,.F.);
#74993=ORIENTED_EDGE('',*,*,#53322,.T.);
#74994=ORIENTED_EDGE('',*,*,#52319,.F.);
#74995=ORIENTED_EDGE('',*,*,#53323,.T.);
#74996=ORIENTED_EDGE('',*,*,#53309,.F.);
#74997=ORIENTED_EDGE('',*,*,#53324,.T.);
#74998=ORIENTED_EDGE('',*,*,#53311,.F.);
#74999=ORIENTED_EDGE('',*,*,#53325,.T.);
#75000=ORIENTED_EDGE('',*,*,#53305,.F.);
#75001=ORIENTED_EDGE('',*,*,#53326,.T.);
#75002=ORIENTED_EDGE('',*,*,#53307,.F.);
#75003=ORIENTED_EDGE('',*,*,#53327,.T.);
#75004=ORIENTED_EDGE('',*,*,#53328,.T.);
#75005=ORIENTED_EDGE('',*,*,#53329,.T.);
#75006=ORIENTED_EDGE('',*,*,#53330,.F.);
#75007=ORIENTED_EDGE('',*,*,#53331,.F.);
#75008=ORIENTED_EDGE('',*,*,#53332,.F.);
#75009=ORIENTED_EDGE('',*,*,#53333,.T.);
#75010=ORIENTED_EDGE('',*,*,#53331,.T.);
#75011=ORIENTED_EDGE('',*,*,#53334,.T.);
#75012=ORIENTED_EDGE('',*,*,#53335,.T.);
#75013=ORIENTED_EDGE('',*,*,#53336,.T.);
#75014=ORIENTED_EDGE('',*,*,#53337,.T.);
#75015=ORIENTED_EDGE('',*,*,#53338,.T.);
#75016=ORIENTED_EDGE('',*,*,#53339,.T.);
#75017=ORIENTED_EDGE('',*,*,#53340,.T.);
#75018=ORIENTED_EDGE('',*,*,#53341,.T.);
#75019=ORIENTED_EDGE('',*,*,#53342,.T.);
#75020=ORIENTED_EDGE('',*,*,#53343,.F.);
#75021=ORIENTED_EDGE('',*,*,#53344,.F.);
#75022=ORIENTED_EDGE('',*,*,#53345,.F.);
#75023=ORIENTED_EDGE('',*,*,#53346,.T.);
#75024=ORIENTED_EDGE('',*,*,#53344,.T.);
#75025=ORIENTED_EDGE('',*,*,#53347,.T.);
#75026=ORIENTED_EDGE('',*,*,#53348,.T.);
#75027=ORIENTED_EDGE('',*,*,#53349,.T.);
#75028=ORIENTED_EDGE('',*,*,#52714,.F.);
#75029=ORIENTED_EDGE('',*,*,#53350,.T.);
#75030=ORIENTED_EDGE('',*,*,#53328,.F.);
#75031=ORIENTED_EDGE('',*,*,#53351,.T.);
#75032=ORIENTED_EDGE('',*,*,#53348,.F.);
#75033=ORIENTED_EDGE('',*,*,#53352,.T.);
#75034=ORIENTED_EDGE('',*,*,#52313,.F.);
#75035=ORIENTED_EDGE('',*,*,#53353,.T.);
#75036=ORIENTED_EDGE('',*,*,#53339,.F.);
#75037=ORIENTED_EDGE('',*,*,#53354,.T.);
#75038=ORIENTED_EDGE('',*,*,#53341,.F.);
#75039=ORIENTED_EDGE('',*,*,#53355,.T.);
#75040=ORIENTED_EDGE('',*,*,#53335,.F.);
#75041=ORIENTED_EDGE('',*,*,#53356,.T.);
#75042=ORIENTED_EDGE('',*,*,#53337,.F.);
#75043=ORIENTED_EDGE('',*,*,#53357,.T.);
#75044=ORIENTED_EDGE('',*,*,#53358,.T.);
#75045=ORIENTED_EDGE('',*,*,#53359,.T.);
#75046=ORIENTED_EDGE('',*,*,#53360,.F.);
#75047=ORIENTED_EDGE('',*,*,#53361,.F.);
#75048=ORIENTED_EDGE('',*,*,#53362,.F.);
#75049=ORIENTED_EDGE('',*,*,#53363,.T.);
#75050=ORIENTED_EDGE('',*,*,#53361,.T.);
#75051=ORIENTED_EDGE('',*,*,#53364,.T.);
#75052=ORIENTED_EDGE('',*,*,#53365,.T.);
#75053=ORIENTED_EDGE('',*,*,#53366,.T.);
#75054=ORIENTED_EDGE('',*,*,#53367,.T.);
#75055=ORIENTED_EDGE('',*,*,#53368,.T.);
#75056=ORIENTED_EDGE('',*,*,#53369,.T.);
#75057=ORIENTED_EDGE('',*,*,#53370,.T.);
#75058=ORIENTED_EDGE('',*,*,#53371,.T.);
#75059=ORIENTED_EDGE('',*,*,#53372,.T.);
#75060=ORIENTED_EDGE('',*,*,#53373,.F.);
#75061=ORIENTED_EDGE('',*,*,#53374,.F.);
#75062=ORIENTED_EDGE('',*,*,#53375,.F.);
#75063=ORIENTED_EDGE('',*,*,#53376,.T.);
#75064=ORIENTED_EDGE('',*,*,#53374,.T.);
#75065=ORIENTED_EDGE('',*,*,#53377,.T.);
#75066=ORIENTED_EDGE('',*,*,#53378,.T.);
#75067=ORIENTED_EDGE('',*,*,#53379,.T.);
#75068=ORIENTED_EDGE('',*,*,#52720,.F.);
#75069=ORIENTED_EDGE('',*,*,#53380,.T.);
#75070=ORIENTED_EDGE('',*,*,#53358,.F.);
#75071=ORIENTED_EDGE('',*,*,#53381,.T.);
#75072=ORIENTED_EDGE('',*,*,#53378,.F.);
#75073=ORIENTED_EDGE('',*,*,#53382,.T.);
#75074=ORIENTED_EDGE('',*,*,#52307,.F.);
#75075=ORIENTED_EDGE('',*,*,#53383,.T.);
#75076=ORIENTED_EDGE('',*,*,#53369,.F.);
#75077=ORIENTED_EDGE('',*,*,#53384,.T.);
#75078=ORIENTED_EDGE('',*,*,#53371,.F.);
#75079=ORIENTED_EDGE('',*,*,#53385,.T.);
#75080=ORIENTED_EDGE('',*,*,#53365,.F.);
#75081=ORIENTED_EDGE('',*,*,#53386,.T.);
#75082=ORIENTED_EDGE('',*,*,#53367,.F.);
#75083=ORIENTED_EDGE('',*,*,#53387,.T.);
#75084=ORIENTED_EDGE('',*,*,#53388,.T.);
#75085=ORIENTED_EDGE('',*,*,#53389,.T.);
#75086=ORIENTED_EDGE('',*,*,#53390,.F.);
#75087=ORIENTED_EDGE('',*,*,#53391,.F.);
#75088=ORIENTED_EDGE('',*,*,#53392,.F.);
#75089=ORIENTED_EDGE('',*,*,#53393,.T.);
#75090=ORIENTED_EDGE('',*,*,#53391,.T.);
#75091=ORIENTED_EDGE('',*,*,#53394,.T.);
#75092=ORIENTED_EDGE('',*,*,#53395,.T.);
#75093=ORIENTED_EDGE('',*,*,#53396,.T.);
#75094=ORIENTED_EDGE('',*,*,#53397,.T.);
#75095=ORIENTED_EDGE('',*,*,#53398,.T.);
#75096=ORIENTED_EDGE('',*,*,#53399,.T.);
#75097=ORIENTED_EDGE('',*,*,#53400,.T.);
#75098=ORIENTED_EDGE('',*,*,#53401,.T.);
#75099=ORIENTED_EDGE('',*,*,#53402,.T.);
#75100=ORIENTED_EDGE('',*,*,#53403,.F.);
#75101=ORIENTED_EDGE('',*,*,#53404,.F.);
#75102=ORIENTED_EDGE('',*,*,#53405,.F.);
#75103=ORIENTED_EDGE('',*,*,#53406,.T.);
#75104=ORIENTED_EDGE('',*,*,#53404,.T.);
#75105=ORIENTED_EDGE('',*,*,#53407,.T.);
#75106=ORIENTED_EDGE('',*,*,#53408,.T.);
#75107=ORIENTED_EDGE('',*,*,#53409,.T.);
#75108=ORIENTED_EDGE('',*,*,#52726,.F.);
#75109=ORIENTED_EDGE('',*,*,#53410,.T.);
#75110=ORIENTED_EDGE('',*,*,#53388,.F.);
#75111=ORIENTED_EDGE('',*,*,#53411,.T.);
#75112=ORIENTED_EDGE('',*,*,#53408,.F.);
#75113=ORIENTED_EDGE('',*,*,#53412,.T.);
#75114=ORIENTED_EDGE('',*,*,#52301,.F.);
#75115=ORIENTED_EDGE('',*,*,#53413,.T.);
#75116=ORIENTED_EDGE('',*,*,#53399,.F.);
#75117=ORIENTED_EDGE('',*,*,#53414,.T.);
#75118=ORIENTED_EDGE('',*,*,#53401,.F.);
#75119=ORIENTED_EDGE('',*,*,#53415,.T.);
#75120=ORIENTED_EDGE('',*,*,#53395,.F.);
#75121=ORIENTED_EDGE('',*,*,#53416,.T.);
#75122=ORIENTED_EDGE('',*,*,#53397,.F.);
#75123=ORIENTED_EDGE('',*,*,#53417,.T.);
#75124=ORIENTED_EDGE('',*,*,#53418,.T.);
#75125=ORIENTED_EDGE('',*,*,#53419,.T.);
#75126=ORIENTED_EDGE('',*,*,#53420,.F.);
#75127=ORIENTED_EDGE('',*,*,#53421,.F.);
#75128=ORIENTED_EDGE('',*,*,#53422,.F.);
#75129=ORIENTED_EDGE('',*,*,#53423,.T.);
#75130=ORIENTED_EDGE('',*,*,#53421,.T.);
#75131=ORIENTED_EDGE('',*,*,#53424,.T.);
#75132=ORIENTED_EDGE('',*,*,#53425,.T.);
#75133=ORIENTED_EDGE('',*,*,#53426,.T.);
#75134=ORIENTED_EDGE('',*,*,#53427,.T.);
#75135=ORIENTED_EDGE('',*,*,#53428,.T.);
#75136=ORIENTED_EDGE('',*,*,#53429,.T.);
#75137=ORIENTED_EDGE('',*,*,#53430,.T.);
#75138=ORIENTED_EDGE('',*,*,#53431,.T.);
#75139=ORIENTED_EDGE('',*,*,#53432,.T.);
#75140=ORIENTED_EDGE('',*,*,#53433,.F.);
#75141=ORIENTED_EDGE('',*,*,#53434,.F.);
#75142=ORIENTED_EDGE('',*,*,#53435,.F.);
#75143=ORIENTED_EDGE('',*,*,#53436,.T.);
#75144=ORIENTED_EDGE('',*,*,#53434,.T.);
#75145=ORIENTED_EDGE('',*,*,#53437,.T.);
#75146=ORIENTED_EDGE('',*,*,#53438,.T.);
#75147=ORIENTED_EDGE('',*,*,#53439,.T.);
#75148=ORIENTED_EDGE('',*,*,#52732,.F.);
#75149=ORIENTED_EDGE('',*,*,#53440,.T.);
#75150=ORIENTED_EDGE('',*,*,#53418,.F.);
#75151=ORIENTED_EDGE('',*,*,#53441,.T.);
#75152=ORIENTED_EDGE('',*,*,#53438,.F.);
#75153=ORIENTED_EDGE('',*,*,#53442,.T.);
#75154=ORIENTED_EDGE('',*,*,#52295,.F.);
#75155=ORIENTED_EDGE('',*,*,#53443,.T.);
#75156=ORIENTED_EDGE('',*,*,#53429,.F.);
#75157=ORIENTED_EDGE('',*,*,#53444,.T.);
#75158=ORIENTED_EDGE('',*,*,#53431,.F.);
#75159=ORIENTED_EDGE('',*,*,#53445,.T.);
#75160=ORIENTED_EDGE('',*,*,#53425,.F.);
#75161=ORIENTED_EDGE('',*,*,#53446,.T.);
#75162=ORIENTED_EDGE('',*,*,#53427,.F.);
#75163=ORIENTED_EDGE('',*,*,#53447,.T.);
#75164=ORIENTED_EDGE('',*,*,#53448,.T.);
#75165=ORIENTED_EDGE('',*,*,#53449,.T.);
#75166=ORIENTED_EDGE('',*,*,#53450,.F.);
#75167=ORIENTED_EDGE('',*,*,#53451,.F.);
#75168=ORIENTED_EDGE('',*,*,#53452,.F.);
#75169=ORIENTED_EDGE('',*,*,#53453,.T.);
#75170=ORIENTED_EDGE('',*,*,#53451,.T.);
#75171=ORIENTED_EDGE('',*,*,#53454,.T.);
#75172=ORIENTED_EDGE('',*,*,#53455,.T.);
#75173=ORIENTED_EDGE('',*,*,#53456,.T.);
#75174=ORIENTED_EDGE('',*,*,#53457,.T.);
#75175=ORIENTED_EDGE('',*,*,#53458,.T.);
#75176=ORIENTED_EDGE('',*,*,#53459,.T.);
#75177=ORIENTED_EDGE('',*,*,#53460,.T.);
#75178=ORIENTED_EDGE('',*,*,#53461,.T.);
#75179=ORIENTED_EDGE('',*,*,#53462,.T.);
#75180=ORIENTED_EDGE('',*,*,#53463,.F.);
#75181=ORIENTED_EDGE('',*,*,#53464,.F.);
#75182=ORIENTED_EDGE('',*,*,#53465,.F.);
#75183=ORIENTED_EDGE('',*,*,#53466,.T.);
#75184=ORIENTED_EDGE('',*,*,#53464,.T.);
#75185=ORIENTED_EDGE('',*,*,#53467,.T.);
#75186=ORIENTED_EDGE('',*,*,#53468,.T.);
#75187=ORIENTED_EDGE('',*,*,#53469,.T.);
#75188=ORIENTED_EDGE('',*,*,#52738,.F.);
#75189=ORIENTED_EDGE('',*,*,#53470,.T.);
#75190=ORIENTED_EDGE('',*,*,#53448,.F.);
#75191=ORIENTED_EDGE('',*,*,#53471,.T.);
#75192=ORIENTED_EDGE('',*,*,#53468,.F.);
#75193=ORIENTED_EDGE('',*,*,#53472,.T.);
#75194=ORIENTED_EDGE('',*,*,#52289,.F.);
#75195=ORIENTED_EDGE('',*,*,#53473,.T.);
#75196=ORIENTED_EDGE('',*,*,#53459,.F.);
#75197=ORIENTED_EDGE('',*,*,#53474,.T.);
#75198=ORIENTED_EDGE('',*,*,#53461,.F.);
#75199=ORIENTED_EDGE('',*,*,#53475,.T.);
#75200=ORIENTED_EDGE('',*,*,#53455,.F.);
#75201=ORIENTED_EDGE('',*,*,#53476,.T.);
#75202=ORIENTED_EDGE('',*,*,#53457,.F.);
#75203=ORIENTED_EDGE('',*,*,#53477,.T.);
#75204=ORIENTED_EDGE('',*,*,#53478,.T.);
#75205=ORIENTED_EDGE('',*,*,#53479,.T.);
#75206=ORIENTED_EDGE('',*,*,#53480,.F.);
#75207=ORIENTED_EDGE('',*,*,#53481,.F.);
#75208=ORIENTED_EDGE('',*,*,#53482,.F.);
#75209=ORIENTED_EDGE('',*,*,#53483,.T.);
#75210=ORIENTED_EDGE('',*,*,#53481,.T.);
#75211=ORIENTED_EDGE('',*,*,#53484,.T.);
#75212=ORIENTED_EDGE('',*,*,#53485,.T.);
#75213=ORIENTED_EDGE('',*,*,#53486,.T.);
#75214=ORIENTED_EDGE('',*,*,#53487,.T.);
#75215=ORIENTED_EDGE('',*,*,#53488,.T.);
#75216=ORIENTED_EDGE('',*,*,#53489,.T.);
#75217=ORIENTED_EDGE('',*,*,#53490,.T.);
#75218=ORIENTED_EDGE('',*,*,#53491,.T.);
#75219=ORIENTED_EDGE('',*,*,#53492,.T.);
#75220=ORIENTED_EDGE('',*,*,#53493,.F.);
#75221=ORIENTED_EDGE('',*,*,#53494,.F.);
#75222=ORIENTED_EDGE('',*,*,#53495,.F.);
#75223=ORIENTED_EDGE('',*,*,#53496,.T.);
#75224=ORIENTED_EDGE('',*,*,#53494,.T.);
#75225=ORIENTED_EDGE('',*,*,#53497,.T.);
#75226=ORIENTED_EDGE('',*,*,#53498,.T.);
#75227=ORIENTED_EDGE('',*,*,#53499,.T.);
#75228=ORIENTED_EDGE('',*,*,#52744,.F.);
#75229=ORIENTED_EDGE('',*,*,#53500,.T.);
#75230=ORIENTED_EDGE('',*,*,#53478,.F.);
#75231=ORIENTED_EDGE('',*,*,#53501,.T.);
#75232=ORIENTED_EDGE('',*,*,#53498,.F.);
#75233=ORIENTED_EDGE('',*,*,#53502,.T.);
#75234=ORIENTED_EDGE('',*,*,#52283,.F.);
#75235=ORIENTED_EDGE('',*,*,#53503,.T.);
#75236=ORIENTED_EDGE('',*,*,#53489,.F.);
#75237=ORIENTED_EDGE('',*,*,#53504,.T.);
#75238=ORIENTED_EDGE('',*,*,#53491,.F.);
#75239=ORIENTED_EDGE('',*,*,#53505,.T.);
#75240=ORIENTED_EDGE('',*,*,#53485,.F.);
#75241=ORIENTED_EDGE('',*,*,#53506,.T.);
#75242=ORIENTED_EDGE('',*,*,#53487,.F.);
#75243=ORIENTED_EDGE('',*,*,#53507,.T.);
#75244=ORIENTED_EDGE('',*,*,#53508,.T.);
#75245=ORIENTED_EDGE('',*,*,#53509,.T.);
#75246=ORIENTED_EDGE('',*,*,#53510,.F.);
#75247=ORIENTED_EDGE('',*,*,#53511,.F.);
#75248=ORIENTED_EDGE('',*,*,#53512,.F.);
#75249=ORIENTED_EDGE('',*,*,#53513,.T.);
#75250=ORIENTED_EDGE('',*,*,#53511,.T.);
#75251=ORIENTED_EDGE('',*,*,#53514,.T.);
#75252=ORIENTED_EDGE('',*,*,#53515,.T.);
#75253=ORIENTED_EDGE('',*,*,#53516,.T.);
#75254=ORIENTED_EDGE('',*,*,#53517,.T.);
#75255=ORIENTED_EDGE('',*,*,#53518,.T.);
#75256=ORIENTED_EDGE('',*,*,#53519,.T.);
#75257=ORIENTED_EDGE('',*,*,#53520,.T.);
#75258=ORIENTED_EDGE('',*,*,#53521,.T.);
#75259=ORIENTED_EDGE('',*,*,#53522,.T.);
#75260=ORIENTED_EDGE('',*,*,#53523,.F.);
#75261=ORIENTED_EDGE('',*,*,#53524,.F.);
#75262=ORIENTED_EDGE('',*,*,#53525,.F.);
#75263=ORIENTED_EDGE('',*,*,#53526,.T.);
#75264=ORIENTED_EDGE('',*,*,#53524,.T.);
#75265=ORIENTED_EDGE('',*,*,#53527,.T.);
#75266=ORIENTED_EDGE('',*,*,#53528,.T.);
#75267=ORIENTED_EDGE('',*,*,#53529,.T.);
#75268=ORIENTED_EDGE('',*,*,#52750,.F.);
#75269=ORIENTED_EDGE('',*,*,#53530,.T.);
#75270=ORIENTED_EDGE('',*,*,#53508,.F.);
#75271=ORIENTED_EDGE('',*,*,#53531,.T.);
#75272=ORIENTED_EDGE('',*,*,#53528,.F.);
#75273=ORIENTED_EDGE('',*,*,#53532,.T.);
#75274=ORIENTED_EDGE('',*,*,#52277,.F.);
#75275=ORIENTED_EDGE('',*,*,#53533,.T.);
#75276=ORIENTED_EDGE('',*,*,#53519,.F.);
#75277=ORIENTED_EDGE('',*,*,#53534,.T.);
#75278=ORIENTED_EDGE('',*,*,#53521,.F.);
#75279=ORIENTED_EDGE('',*,*,#53535,.T.);
#75280=ORIENTED_EDGE('',*,*,#53515,.F.);
#75281=ORIENTED_EDGE('',*,*,#53536,.T.);
#75282=ORIENTED_EDGE('',*,*,#53517,.F.);
#75283=ORIENTED_EDGE('',*,*,#53537,.T.);
#75284=ORIENTED_EDGE('',*,*,#53538,.T.);
#75285=ORIENTED_EDGE('',*,*,#53539,.T.);
#75286=ORIENTED_EDGE('',*,*,#53540,.F.);
#75287=ORIENTED_EDGE('',*,*,#53541,.F.);
#75288=ORIENTED_EDGE('',*,*,#53542,.F.);
#75289=ORIENTED_EDGE('',*,*,#53543,.T.);
#75290=ORIENTED_EDGE('',*,*,#53541,.T.);
#75291=ORIENTED_EDGE('',*,*,#53544,.T.);
#75292=ORIENTED_EDGE('',*,*,#53545,.T.);
#75293=ORIENTED_EDGE('',*,*,#53546,.T.);
#75294=ORIENTED_EDGE('',*,*,#53547,.T.);
#75295=ORIENTED_EDGE('',*,*,#53548,.T.);
#75296=ORIENTED_EDGE('',*,*,#53549,.T.);
#75297=ORIENTED_EDGE('',*,*,#53550,.T.);
#75298=ORIENTED_EDGE('',*,*,#53551,.T.);
#75299=ORIENTED_EDGE('',*,*,#53552,.T.);
#75300=ORIENTED_EDGE('',*,*,#53553,.F.);
#75301=ORIENTED_EDGE('',*,*,#53554,.F.);
#75302=ORIENTED_EDGE('',*,*,#53555,.F.);
#75303=ORIENTED_EDGE('',*,*,#53556,.T.);
#75304=ORIENTED_EDGE('',*,*,#53554,.T.);
#75305=ORIENTED_EDGE('',*,*,#53557,.T.);
#75306=ORIENTED_EDGE('',*,*,#53558,.T.);
#75307=ORIENTED_EDGE('',*,*,#53559,.T.);
#75308=ORIENTED_EDGE('',*,*,#52756,.F.);
#75309=ORIENTED_EDGE('',*,*,#53560,.T.);
#75310=ORIENTED_EDGE('',*,*,#53538,.F.);
#75311=ORIENTED_EDGE('',*,*,#53561,.T.);
#75312=ORIENTED_EDGE('',*,*,#53558,.F.);
#75313=ORIENTED_EDGE('',*,*,#53562,.T.);
#75314=ORIENTED_EDGE('',*,*,#52271,.F.);
#75315=ORIENTED_EDGE('',*,*,#53563,.T.);
#75316=ORIENTED_EDGE('',*,*,#53549,.F.);
#75317=ORIENTED_EDGE('',*,*,#53564,.T.);
#75318=ORIENTED_EDGE('',*,*,#53551,.F.);
#75319=ORIENTED_EDGE('',*,*,#53565,.T.);
#75320=ORIENTED_EDGE('',*,*,#53545,.F.);
#75321=ORIENTED_EDGE('',*,*,#53566,.T.);
#75322=ORIENTED_EDGE('',*,*,#53547,.F.);
#75323=ORIENTED_EDGE('',*,*,#53567,.T.);
#75324=ORIENTED_EDGE('',*,*,#53568,.T.);
#75325=ORIENTED_EDGE('',*,*,#53569,.T.);
#75326=ORIENTED_EDGE('',*,*,#53570,.F.);
#75327=ORIENTED_EDGE('',*,*,#53571,.F.);
#75328=ORIENTED_EDGE('',*,*,#53572,.F.);
#75329=ORIENTED_EDGE('',*,*,#53573,.T.);
#75330=ORIENTED_EDGE('',*,*,#53571,.T.);
#75331=ORIENTED_EDGE('',*,*,#53574,.T.);
#75332=ORIENTED_EDGE('',*,*,#53575,.T.);
#75333=ORIENTED_EDGE('',*,*,#53576,.T.);
#75334=ORIENTED_EDGE('',*,*,#53577,.T.);
#75335=ORIENTED_EDGE('',*,*,#53578,.T.);
#75336=ORIENTED_EDGE('',*,*,#53579,.T.);
#75337=ORIENTED_EDGE('',*,*,#53580,.T.);
#75338=ORIENTED_EDGE('',*,*,#53581,.T.);
#75339=ORIENTED_EDGE('',*,*,#53582,.T.);
#75340=ORIENTED_EDGE('',*,*,#53583,.F.);
#75341=ORIENTED_EDGE('',*,*,#53584,.F.);
#75342=ORIENTED_EDGE('',*,*,#53585,.F.);
#75343=ORIENTED_EDGE('',*,*,#53586,.T.);
#75344=ORIENTED_EDGE('',*,*,#53584,.T.);
#75345=ORIENTED_EDGE('',*,*,#53587,.T.);
#75346=ORIENTED_EDGE('',*,*,#53588,.T.);
#75347=ORIENTED_EDGE('',*,*,#53589,.T.);
#75348=ORIENTED_EDGE('',*,*,#52762,.F.);
#75349=ORIENTED_EDGE('',*,*,#53590,.T.);
#75350=ORIENTED_EDGE('',*,*,#53568,.F.);
#75351=ORIENTED_EDGE('',*,*,#53591,.T.);
#75352=ORIENTED_EDGE('',*,*,#53588,.F.);
#75353=ORIENTED_EDGE('',*,*,#53592,.T.);
#75354=ORIENTED_EDGE('',*,*,#52265,.F.);
#75355=ORIENTED_EDGE('',*,*,#53593,.T.);
#75356=ORIENTED_EDGE('',*,*,#53579,.F.);
#75357=ORIENTED_EDGE('',*,*,#53594,.T.);
#75358=ORIENTED_EDGE('',*,*,#53581,.F.);
#75359=ORIENTED_EDGE('',*,*,#53595,.T.);
#75360=ORIENTED_EDGE('',*,*,#53575,.F.);
#75361=ORIENTED_EDGE('',*,*,#53596,.T.);
#75362=ORIENTED_EDGE('',*,*,#53577,.F.);
#75363=ORIENTED_EDGE('',*,*,#53597,.T.);
#75364=ORIENTED_EDGE('',*,*,#53598,.T.);
#75365=ORIENTED_EDGE('',*,*,#53599,.T.);
#75366=ORIENTED_EDGE('',*,*,#53600,.F.);
#75367=ORIENTED_EDGE('',*,*,#53601,.F.);
#75368=ORIENTED_EDGE('',*,*,#53602,.F.);
#75369=ORIENTED_EDGE('',*,*,#53603,.T.);
#75370=ORIENTED_EDGE('',*,*,#53601,.T.);
#75371=ORIENTED_EDGE('',*,*,#53604,.T.);
#75372=ORIENTED_EDGE('',*,*,#53605,.T.);
#75373=ORIENTED_EDGE('',*,*,#53606,.T.);
#75374=ORIENTED_EDGE('',*,*,#53607,.T.);
#75375=ORIENTED_EDGE('',*,*,#53608,.T.);
#75376=ORIENTED_EDGE('',*,*,#53609,.T.);
#75377=ORIENTED_EDGE('',*,*,#53610,.T.);
#75378=ORIENTED_EDGE('',*,*,#53611,.T.);
#75379=ORIENTED_EDGE('',*,*,#53612,.T.);
#75380=ORIENTED_EDGE('',*,*,#53613,.F.);
#75381=ORIENTED_EDGE('',*,*,#53614,.F.);
#75382=ORIENTED_EDGE('',*,*,#53615,.F.);
#75383=ORIENTED_EDGE('',*,*,#53616,.T.);
#75384=ORIENTED_EDGE('',*,*,#53614,.T.);
#75385=ORIENTED_EDGE('',*,*,#53617,.T.);
#75386=ORIENTED_EDGE('',*,*,#53618,.T.);
#75387=ORIENTED_EDGE('',*,*,#53619,.T.);
#75388=ORIENTED_EDGE('',*,*,#52768,.F.);
#75389=ORIENTED_EDGE('',*,*,#53620,.T.);
#75390=ORIENTED_EDGE('',*,*,#53598,.F.);
#75391=ORIENTED_EDGE('',*,*,#53621,.T.);
#75392=ORIENTED_EDGE('',*,*,#53618,.F.);
#75393=ORIENTED_EDGE('',*,*,#53622,.T.);
#75394=ORIENTED_EDGE('',*,*,#52259,.F.);
#75395=ORIENTED_EDGE('',*,*,#53623,.T.);
#75396=ORIENTED_EDGE('',*,*,#53609,.F.);
#75397=ORIENTED_EDGE('',*,*,#53624,.T.);
#75398=ORIENTED_EDGE('',*,*,#53611,.F.);
#75399=ORIENTED_EDGE('',*,*,#53625,.T.);
#75400=ORIENTED_EDGE('',*,*,#53605,.F.);
#75401=ORIENTED_EDGE('',*,*,#53626,.T.);
#75402=ORIENTED_EDGE('',*,*,#53607,.F.);
#75403=ORIENTED_EDGE('',*,*,#53627,.T.);
#75404=ORIENTED_EDGE('',*,*,#53628,.T.);
#75405=ORIENTED_EDGE('',*,*,#53629,.T.);
#75406=ORIENTED_EDGE('',*,*,#53630,.F.);
#75407=ORIENTED_EDGE('',*,*,#53631,.F.);
#75408=ORIENTED_EDGE('',*,*,#53632,.F.);
#75409=ORIENTED_EDGE('',*,*,#53633,.T.);
#75410=ORIENTED_EDGE('',*,*,#53631,.T.);
#75411=ORIENTED_EDGE('',*,*,#53634,.T.);
#75412=ORIENTED_EDGE('',*,*,#53635,.T.);
#75413=ORIENTED_EDGE('',*,*,#53636,.T.);
#75414=ORIENTED_EDGE('',*,*,#53637,.T.);
#75415=ORIENTED_EDGE('',*,*,#53638,.T.);
#75416=ORIENTED_EDGE('',*,*,#53639,.T.);
#75417=ORIENTED_EDGE('',*,*,#53640,.T.);
#75418=ORIENTED_EDGE('',*,*,#53641,.T.);
#75419=ORIENTED_EDGE('',*,*,#53642,.T.);
#75420=ORIENTED_EDGE('',*,*,#53643,.F.);
#75421=ORIENTED_EDGE('',*,*,#53644,.F.);
#75422=ORIENTED_EDGE('',*,*,#53645,.F.);
#75423=ORIENTED_EDGE('',*,*,#53646,.T.);
#75424=ORIENTED_EDGE('',*,*,#53644,.T.);
#75425=ORIENTED_EDGE('',*,*,#53647,.T.);
#75426=ORIENTED_EDGE('',*,*,#53648,.T.);
#75427=ORIENTED_EDGE('',*,*,#53649,.T.);
#75428=ORIENTED_EDGE('',*,*,#52774,.F.);
#75429=ORIENTED_EDGE('',*,*,#53650,.T.);
#75430=ORIENTED_EDGE('',*,*,#53628,.F.);
#75431=ORIENTED_EDGE('',*,*,#53651,.T.);
#75432=ORIENTED_EDGE('',*,*,#53648,.F.);
#75433=ORIENTED_EDGE('',*,*,#53652,.T.);
#75434=ORIENTED_EDGE('',*,*,#52253,.F.);
#75435=ORIENTED_EDGE('',*,*,#53653,.T.);
#75436=ORIENTED_EDGE('',*,*,#53639,.F.);
#75437=ORIENTED_EDGE('',*,*,#53654,.T.);
#75438=ORIENTED_EDGE('',*,*,#53641,.F.);
#75439=ORIENTED_EDGE('',*,*,#53655,.T.);
#75440=ORIENTED_EDGE('',*,*,#53635,.F.);
#75441=ORIENTED_EDGE('',*,*,#53656,.T.);
#75442=ORIENTED_EDGE('',*,*,#53637,.F.);
#75443=ORIENTED_EDGE('',*,*,#53657,.T.);
#75444=ORIENTED_EDGE('',*,*,#53658,.T.);
#75445=ORIENTED_EDGE('',*,*,#53659,.T.);
#75446=ORIENTED_EDGE('',*,*,#53660,.F.);
#75447=ORIENTED_EDGE('',*,*,#53661,.F.);
#75448=ORIENTED_EDGE('',*,*,#53662,.F.);
#75449=ORIENTED_EDGE('',*,*,#53663,.T.);
#75450=ORIENTED_EDGE('',*,*,#53661,.T.);
#75451=ORIENTED_EDGE('',*,*,#53664,.T.);
#75452=ORIENTED_EDGE('',*,*,#53665,.T.);
#75453=ORIENTED_EDGE('',*,*,#53666,.T.);
#75454=ORIENTED_EDGE('',*,*,#53667,.T.);
#75455=ORIENTED_EDGE('',*,*,#53668,.T.);
#75456=ORIENTED_EDGE('',*,*,#53669,.T.);
#75457=ORIENTED_EDGE('',*,*,#53670,.T.);
#75458=ORIENTED_EDGE('',*,*,#53671,.T.);
#75459=ORIENTED_EDGE('',*,*,#53672,.T.);
#75460=ORIENTED_EDGE('',*,*,#53673,.F.);
#75461=ORIENTED_EDGE('',*,*,#53674,.F.);
#75462=ORIENTED_EDGE('',*,*,#53675,.F.);
#75463=ORIENTED_EDGE('',*,*,#53676,.T.);
#75464=ORIENTED_EDGE('',*,*,#53674,.T.);
#75465=ORIENTED_EDGE('',*,*,#53677,.T.);
#75466=ORIENTED_EDGE('',*,*,#53678,.T.);
#75467=ORIENTED_EDGE('',*,*,#53679,.T.);
#75468=ORIENTED_EDGE('',*,*,#52780,.F.);
#75469=ORIENTED_EDGE('',*,*,#53680,.T.);
#75470=ORIENTED_EDGE('',*,*,#53658,.F.);
#75471=ORIENTED_EDGE('',*,*,#53681,.T.);
#75472=ORIENTED_EDGE('',*,*,#53678,.F.);
#75473=ORIENTED_EDGE('',*,*,#53682,.T.);
#75474=ORIENTED_EDGE('',*,*,#52247,.F.);
#75475=ORIENTED_EDGE('',*,*,#53683,.T.);
#75476=ORIENTED_EDGE('',*,*,#53669,.F.);
#75477=ORIENTED_EDGE('',*,*,#53684,.T.);
#75478=ORIENTED_EDGE('',*,*,#53671,.F.);
#75479=ORIENTED_EDGE('',*,*,#53685,.T.);
#75480=ORIENTED_EDGE('',*,*,#53665,.F.);
#75481=ORIENTED_EDGE('',*,*,#53686,.T.);
#75482=ORIENTED_EDGE('',*,*,#53667,.F.);
#75483=ORIENTED_EDGE('',*,*,#53687,.T.);
#75484=ORIENTED_EDGE('',*,*,#53688,.T.);
#75485=ORIENTED_EDGE('',*,*,#53689,.T.);
#75486=ORIENTED_EDGE('',*,*,#53690,.F.);
#75487=ORIENTED_EDGE('',*,*,#53691,.F.);
#75488=ORIENTED_EDGE('',*,*,#53692,.F.);
#75489=ORIENTED_EDGE('',*,*,#53693,.T.);
#75490=ORIENTED_EDGE('',*,*,#53691,.T.);
#75491=ORIENTED_EDGE('',*,*,#53694,.T.);
#75492=ORIENTED_EDGE('',*,*,#53695,.T.);
#75493=ORIENTED_EDGE('',*,*,#53696,.T.);
#75494=ORIENTED_EDGE('',*,*,#53697,.T.);
#75495=ORIENTED_EDGE('',*,*,#53698,.T.);
#75496=ORIENTED_EDGE('',*,*,#53699,.T.);
#75497=ORIENTED_EDGE('',*,*,#53700,.T.);
#75498=ORIENTED_EDGE('',*,*,#53701,.T.);
#75499=ORIENTED_EDGE('',*,*,#53702,.T.);
#75500=ORIENTED_EDGE('',*,*,#53703,.F.);
#75501=ORIENTED_EDGE('',*,*,#53704,.F.);
#75502=ORIENTED_EDGE('',*,*,#53705,.F.);
#75503=ORIENTED_EDGE('',*,*,#53706,.T.);
#75504=ORIENTED_EDGE('',*,*,#53704,.T.);
#75505=ORIENTED_EDGE('',*,*,#53707,.T.);
#75506=ORIENTED_EDGE('',*,*,#53708,.T.);
#75507=ORIENTED_EDGE('',*,*,#53709,.T.);
#75508=ORIENTED_EDGE('',*,*,#52425,.F.);
#75509=ORIENTED_EDGE('',*,*,#53710,.T.);
#75510=ORIENTED_EDGE('',*,*,#53688,.F.);
#75511=ORIENTED_EDGE('',*,*,#53711,.T.);
#75512=ORIENTED_EDGE('',*,*,#53708,.F.);
#75513=ORIENTED_EDGE('',*,*,#53712,.T.);
#75514=ORIENTED_EDGE('',*,*,#52241,.F.);
#75515=ORIENTED_EDGE('',*,*,#53713,.T.);
#75516=ORIENTED_EDGE('',*,*,#53699,.F.);
#75517=ORIENTED_EDGE('',*,*,#53714,.T.);
#75518=ORIENTED_EDGE('',*,*,#53701,.F.);
#75519=ORIENTED_EDGE('',*,*,#53715,.T.);
#75520=ORIENTED_EDGE('',*,*,#53695,.F.);
#75521=ORIENTED_EDGE('',*,*,#53716,.T.);
#75522=ORIENTED_EDGE('',*,*,#53697,.F.);
#75523=ORIENTED_EDGE('',*,*,#53717,.T.);
#75524=ORIENTED_EDGE('',*,*,#53718,.T.);
#75525=ORIENTED_EDGE('',*,*,#53719,.T.);
#75526=ORIENTED_EDGE('',*,*,#53720,.F.);
#75527=ORIENTED_EDGE('',*,*,#53721,.F.);
#75528=ORIENTED_EDGE('',*,*,#53722,.F.);
#75529=ORIENTED_EDGE('',*,*,#53723,.T.);
#75530=ORIENTED_EDGE('',*,*,#53721,.T.);
#75531=ORIENTED_EDGE('',*,*,#53724,.T.);
#75532=ORIENTED_EDGE('',*,*,#53725,.T.);
#75533=ORIENTED_EDGE('',*,*,#53726,.T.);
#75534=ORIENTED_EDGE('',*,*,#53727,.T.);
#75535=ORIENTED_EDGE('',*,*,#53728,.T.);
#75536=ORIENTED_EDGE('',*,*,#53729,.T.);
#75537=ORIENTED_EDGE('',*,*,#53730,.T.);
#75538=ORIENTED_EDGE('',*,*,#53731,.T.);
#75539=ORIENTED_EDGE('',*,*,#53732,.T.);
#75540=ORIENTED_EDGE('',*,*,#53733,.F.);
#75541=ORIENTED_EDGE('',*,*,#53734,.F.);
#75542=ORIENTED_EDGE('',*,*,#53735,.F.);
#75543=ORIENTED_EDGE('',*,*,#53736,.T.);
#75544=ORIENTED_EDGE('',*,*,#53734,.T.);
#75545=ORIENTED_EDGE('',*,*,#53737,.T.);
#75546=ORIENTED_EDGE('',*,*,#53738,.T.);
#75547=ORIENTED_EDGE('',*,*,#53739,.T.);
#75548=ORIENTED_EDGE('',*,*,#52431,.F.);
#75549=ORIENTED_EDGE('',*,*,#53740,.T.);
#75550=ORIENTED_EDGE('',*,*,#53718,.F.);
#75551=ORIENTED_EDGE('',*,*,#53741,.T.);
#75552=ORIENTED_EDGE('',*,*,#53738,.F.);
#75553=ORIENTED_EDGE('',*,*,#53742,.T.);
#75554=ORIENTED_EDGE('',*,*,#52235,.F.);
#75555=ORIENTED_EDGE('',*,*,#53743,.T.);
#75556=ORIENTED_EDGE('',*,*,#53729,.F.);
#75557=ORIENTED_EDGE('',*,*,#53744,.T.);
#75558=ORIENTED_EDGE('',*,*,#53731,.F.);
#75559=ORIENTED_EDGE('',*,*,#53745,.T.);
#75560=ORIENTED_EDGE('',*,*,#53725,.F.);
#75561=ORIENTED_EDGE('',*,*,#53746,.T.);
#75562=ORIENTED_EDGE('',*,*,#53727,.F.);
#75563=ORIENTED_EDGE('',*,*,#53747,.T.);
#75564=ORIENTED_EDGE('',*,*,#53748,.T.);
#75565=ORIENTED_EDGE('',*,*,#53749,.T.);
#75566=ORIENTED_EDGE('',*,*,#53750,.F.);
#75567=ORIENTED_EDGE('',*,*,#53751,.F.);
#75568=ORIENTED_EDGE('',*,*,#53752,.F.);
#75569=ORIENTED_EDGE('',*,*,#53753,.T.);
#75570=ORIENTED_EDGE('',*,*,#53751,.T.);
#75571=ORIENTED_EDGE('',*,*,#53754,.T.);
#75572=ORIENTED_EDGE('',*,*,#53755,.T.);
#75573=ORIENTED_EDGE('',*,*,#53756,.T.);
#75574=ORIENTED_EDGE('',*,*,#53757,.T.);
#75575=ORIENTED_EDGE('',*,*,#53758,.T.);
#75576=ORIENTED_EDGE('',*,*,#53759,.T.);
#75577=ORIENTED_EDGE('',*,*,#53760,.T.);
#75578=ORIENTED_EDGE('',*,*,#53761,.T.);
#75579=ORIENTED_EDGE('',*,*,#53762,.T.);
#75580=ORIENTED_EDGE('',*,*,#53763,.F.);
#75581=ORIENTED_EDGE('',*,*,#53764,.F.);
#75582=ORIENTED_EDGE('',*,*,#53765,.F.);
#75583=ORIENTED_EDGE('',*,*,#53766,.T.);
#75584=ORIENTED_EDGE('',*,*,#53764,.T.);
#75585=ORIENTED_EDGE('',*,*,#53767,.T.);
#75586=ORIENTED_EDGE('',*,*,#53768,.T.);
#75587=ORIENTED_EDGE('',*,*,#53769,.T.);
#75588=ORIENTED_EDGE('',*,*,#52437,.F.);
#75589=ORIENTED_EDGE('',*,*,#53770,.T.);
#75590=ORIENTED_EDGE('',*,*,#53748,.F.);
#75591=ORIENTED_EDGE('',*,*,#53771,.T.);
#75592=ORIENTED_EDGE('',*,*,#53768,.F.);
#75593=ORIENTED_EDGE('',*,*,#53772,.T.);
#75594=ORIENTED_EDGE('',*,*,#52229,.F.);
#75595=ORIENTED_EDGE('',*,*,#53773,.T.);
#75596=ORIENTED_EDGE('',*,*,#53759,.F.);
#75597=ORIENTED_EDGE('',*,*,#53774,.T.);
#75598=ORIENTED_EDGE('',*,*,#53761,.F.);
#75599=ORIENTED_EDGE('',*,*,#53775,.T.);
#75600=ORIENTED_EDGE('',*,*,#53755,.F.);
#75601=ORIENTED_EDGE('',*,*,#53776,.T.);
#75602=ORIENTED_EDGE('',*,*,#53757,.F.);
#75603=ORIENTED_EDGE('',*,*,#53777,.T.);
#75604=ORIENTED_EDGE('',*,*,#53778,.T.);
#75605=ORIENTED_EDGE('',*,*,#53779,.T.);
#75606=ORIENTED_EDGE('',*,*,#53780,.F.);
#75607=ORIENTED_EDGE('',*,*,#53781,.F.);
#75608=ORIENTED_EDGE('',*,*,#53782,.F.);
#75609=ORIENTED_EDGE('',*,*,#53783,.T.);
#75610=ORIENTED_EDGE('',*,*,#53781,.T.);
#75611=ORIENTED_EDGE('',*,*,#53784,.T.);
#75612=ORIENTED_EDGE('',*,*,#53785,.T.);
#75613=ORIENTED_EDGE('',*,*,#53786,.T.);
#75614=ORIENTED_EDGE('',*,*,#53787,.T.);
#75615=ORIENTED_EDGE('',*,*,#53788,.T.);
#75616=ORIENTED_EDGE('',*,*,#53789,.T.);
#75617=ORIENTED_EDGE('',*,*,#53790,.T.);
#75618=ORIENTED_EDGE('',*,*,#53791,.T.);
#75619=ORIENTED_EDGE('',*,*,#53792,.T.);
#75620=ORIENTED_EDGE('',*,*,#53793,.F.);
#75621=ORIENTED_EDGE('',*,*,#53794,.F.);
#75622=ORIENTED_EDGE('',*,*,#53795,.F.);
#75623=ORIENTED_EDGE('',*,*,#53796,.T.);
#75624=ORIENTED_EDGE('',*,*,#53794,.T.);
#75625=ORIENTED_EDGE('',*,*,#53797,.T.);
#75626=ORIENTED_EDGE('',*,*,#53798,.T.);
#75627=ORIENTED_EDGE('',*,*,#53799,.T.);
#75628=ORIENTED_EDGE('',*,*,#52443,.F.);
#75629=ORIENTED_EDGE('',*,*,#53800,.T.);
#75630=ORIENTED_EDGE('',*,*,#53778,.F.);
#75631=ORIENTED_EDGE('',*,*,#53801,.T.);
#75632=ORIENTED_EDGE('',*,*,#53798,.F.);
#75633=ORIENTED_EDGE('',*,*,#53802,.T.);
#75634=ORIENTED_EDGE('',*,*,#52223,.F.);
#75635=ORIENTED_EDGE('',*,*,#53803,.T.);
#75636=ORIENTED_EDGE('',*,*,#53789,.F.);
#75637=ORIENTED_EDGE('',*,*,#53804,.T.);
#75638=ORIENTED_EDGE('',*,*,#53791,.F.);
#75639=ORIENTED_EDGE('',*,*,#53805,.T.);
#75640=ORIENTED_EDGE('',*,*,#53785,.F.);
#75641=ORIENTED_EDGE('',*,*,#53806,.T.);
#75642=ORIENTED_EDGE('',*,*,#53787,.F.);
#75643=ORIENTED_EDGE('',*,*,#53807,.T.);
#75644=ORIENTED_EDGE('',*,*,#53808,.T.);
#75645=ORIENTED_EDGE('',*,*,#53809,.T.);
#75646=ORIENTED_EDGE('',*,*,#53810,.F.);
#75647=ORIENTED_EDGE('',*,*,#53811,.F.);
#75648=ORIENTED_EDGE('',*,*,#53812,.F.);
#75649=ORIENTED_EDGE('',*,*,#53813,.T.);
#75650=ORIENTED_EDGE('',*,*,#53811,.T.);
#75651=ORIENTED_EDGE('',*,*,#53814,.T.);
#75652=ORIENTED_EDGE('',*,*,#53815,.T.);
#75653=ORIENTED_EDGE('',*,*,#53816,.T.);
#75654=ORIENTED_EDGE('',*,*,#53817,.T.);
#75655=ORIENTED_EDGE('',*,*,#53818,.T.);
#75656=ORIENTED_EDGE('',*,*,#53819,.T.);
#75657=ORIENTED_EDGE('',*,*,#53820,.T.);
#75658=ORIENTED_EDGE('',*,*,#53821,.T.);
#75659=ORIENTED_EDGE('',*,*,#53822,.T.);
#75660=ORIENTED_EDGE('',*,*,#53823,.F.);
#75661=ORIENTED_EDGE('',*,*,#53824,.F.);
#75662=ORIENTED_EDGE('',*,*,#53825,.F.);
#75663=ORIENTED_EDGE('',*,*,#53826,.T.);
#75664=ORIENTED_EDGE('',*,*,#53824,.T.);
#75665=ORIENTED_EDGE('',*,*,#53827,.T.);
#75666=ORIENTED_EDGE('',*,*,#53828,.T.);
#75667=ORIENTED_EDGE('',*,*,#53829,.T.);
#75668=ORIENTED_EDGE('',*,*,#52449,.F.);
#75669=ORIENTED_EDGE('',*,*,#53830,.T.);
#75670=ORIENTED_EDGE('',*,*,#53808,.F.);
#75671=ORIENTED_EDGE('',*,*,#53831,.T.);
#75672=ORIENTED_EDGE('',*,*,#53828,.F.);
#75673=ORIENTED_EDGE('',*,*,#53832,.T.);
#75674=ORIENTED_EDGE('',*,*,#52217,.F.);
#75675=ORIENTED_EDGE('',*,*,#53833,.T.);
#75676=ORIENTED_EDGE('',*,*,#53819,.F.);
#75677=ORIENTED_EDGE('',*,*,#53834,.T.);
#75678=ORIENTED_EDGE('',*,*,#53821,.F.);
#75679=ORIENTED_EDGE('',*,*,#53835,.T.);
#75680=ORIENTED_EDGE('',*,*,#53815,.F.);
#75681=ORIENTED_EDGE('',*,*,#53836,.T.);
#75682=ORIENTED_EDGE('',*,*,#53817,.F.);
#75683=ORIENTED_EDGE('',*,*,#53837,.T.);
#75684=ORIENTED_EDGE('',*,*,#53838,.T.);
#75685=ORIENTED_EDGE('',*,*,#53839,.T.);
#75686=ORIENTED_EDGE('',*,*,#53840,.F.);
#75687=ORIENTED_EDGE('',*,*,#53841,.F.);
#75688=ORIENTED_EDGE('',*,*,#53842,.F.);
#75689=ORIENTED_EDGE('',*,*,#53843,.T.);
#75690=ORIENTED_EDGE('',*,*,#53841,.T.);
#75691=ORIENTED_EDGE('',*,*,#53844,.T.);
#75692=ORIENTED_EDGE('',*,*,#53845,.T.);
#75693=ORIENTED_EDGE('',*,*,#53846,.T.);
#75694=ORIENTED_EDGE('',*,*,#53847,.T.);
#75695=ORIENTED_EDGE('',*,*,#53848,.T.);
#75696=ORIENTED_EDGE('',*,*,#53849,.T.);
#75697=ORIENTED_EDGE('',*,*,#53850,.T.);
#75698=ORIENTED_EDGE('',*,*,#53851,.T.);
#75699=ORIENTED_EDGE('',*,*,#53852,.T.);
#75700=ORIENTED_EDGE('',*,*,#53853,.F.);
#75701=ORIENTED_EDGE('',*,*,#53854,.F.);
#75702=ORIENTED_EDGE('',*,*,#53855,.F.);
#75703=ORIENTED_EDGE('',*,*,#53856,.T.);
#75704=ORIENTED_EDGE('',*,*,#53854,.T.);
#75705=ORIENTED_EDGE('',*,*,#53857,.T.);
#75706=ORIENTED_EDGE('',*,*,#53858,.T.);
#75707=ORIENTED_EDGE('',*,*,#53859,.T.);
#75708=ORIENTED_EDGE('',*,*,#52455,.F.);
#75709=ORIENTED_EDGE('',*,*,#53860,.T.);
#75710=ORIENTED_EDGE('',*,*,#53838,.F.);
#75711=ORIENTED_EDGE('',*,*,#53861,.T.);
#75712=ORIENTED_EDGE('',*,*,#53858,.F.);
#75713=ORIENTED_EDGE('',*,*,#53862,.T.);
#75714=ORIENTED_EDGE('',*,*,#52211,.F.);
#75715=ORIENTED_EDGE('',*,*,#53863,.T.);
#75716=ORIENTED_EDGE('',*,*,#53849,.F.);
#75717=ORIENTED_EDGE('',*,*,#53864,.T.);
#75718=ORIENTED_EDGE('',*,*,#53851,.F.);
#75719=ORIENTED_EDGE('',*,*,#53865,.T.);
#75720=ORIENTED_EDGE('',*,*,#53845,.F.);
#75721=ORIENTED_EDGE('',*,*,#53866,.T.);
#75722=ORIENTED_EDGE('',*,*,#53847,.F.);
#75723=ORIENTED_EDGE('',*,*,#53867,.T.);
#75724=ORIENTED_EDGE('',*,*,#53868,.T.);
#75725=ORIENTED_EDGE('',*,*,#53869,.T.);
#75726=ORIENTED_EDGE('',*,*,#53870,.F.);
#75727=ORIENTED_EDGE('',*,*,#53871,.F.);
#75728=ORIENTED_EDGE('',*,*,#53872,.F.);
#75729=ORIENTED_EDGE('',*,*,#53873,.T.);
#75730=ORIENTED_EDGE('',*,*,#53871,.T.);
#75731=ORIENTED_EDGE('',*,*,#53874,.T.);
#75732=ORIENTED_EDGE('',*,*,#53875,.T.);
#75733=ORIENTED_EDGE('',*,*,#53876,.T.);
#75734=ORIENTED_EDGE('',*,*,#53877,.T.);
#75735=ORIENTED_EDGE('',*,*,#53878,.T.);
#75736=ORIENTED_EDGE('',*,*,#53879,.T.);
#75737=ORIENTED_EDGE('',*,*,#53880,.T.);
#75738=ORIENTED_EDGE('',*,*,#53881,.T.);
#75739=ORIENTED_EDGE('',*,*,#53882,.T.);
#75740=ORIENTED_EDGE('',*,*,#53883,.F.);
#75741=ORIENTED_EDGE('',*,*,#53884,.F.);
#75742=ORIENTED_EDGE('',*,*,#53885,.F.);
#75743=ORIENTED_EDGE('',*,*,#53886,.T.);
#75744=ORIENTED_EDGE('',*,*,#53884,.T.);
#75745=ORIENTED_EDGE('',*,*,#53887,.T.);
#75746=ORIENTED_EDGE('',*,*,#53888,.T.);
#75747=ORIENTED_EDGE('',*,*,#53889,.T.);
#75748=ORIENTED_EDGE('',*,*,#52461,.F.);
#75749=ORIENTED_EDGE('',*,*,#53890,.T.);
#75750=ORIENTED_EDGE('',*,*,#53868,.F.);
#75751=ORIENTED_EDGE('',*,*,#53891,.T.);
#75752=ORIENTED_EDGE('',*,*,#53888,.F.);
#75753=ORIENTED_EDGE('',*,*,#53892,.T.);
#75754=ORIENTED_EDGE('',*,*,#52205,.F.);
#75755=ORIENTED_EDGE('',*,*,#53893,.T.);
#75756=ORIENTED_EDGE('',*,*,#53879,.F.);
#75757=ORIENTED_EDGE('',*,*,#53894,.T.);
#75758=ORIENTED_EDGE('',*,*,#53881,.F.);
#75759=ORIENTED_EDGE('',*,*,#53895,.T.);
#75760=ORIENTED_EDGE('',*,*,#53875,.F.);
#75761=ORIENTED_EDGE('',*,*,#53896,.T.);
#75762=ORIENTED_EDGE('',*,*,#53877,.F.);
#75763=ORIENTED_EDGE('',*,*,#53897,.T.);
#75764=ORIENTED_EDGE('',*,*,#53898,.T.);
#75765=ORIENTED_EDGE('',*,*,#53899,.T.);
#75766=ORIENTED_EDGE('',*,*,#53900,.F.);
#75767=ORIENTED_EDGE('',*,*,#53901,.F.);
#75768=ORIENTED_EDGE('',*,*,#53902,.F.);
#75769=ORIENTED_EDGE('',*,*,#53903,.T.);
#75770=ORIENTED_EDGE('',*,*,#53901,.T.);
#75771=ORIENTED_EDGE('',*,*,#53904,.T.);
#75772=ORIENTED_EDGE('',*,*,#53905,.T.);
#75773=ORIENTED_EDGE('',*,*,#53906,.T.);
#75774=ORIENTED_EDGE('',*,*,#53907,.T.);
#75775=ORIENTED_EDGE('',*,*,#53908,.T.);
#75776=ORIENTED_EDGE('',*,*,#53909,.T.);
#75777=ORIENTED_EDGE('',*,*,#53910,.T.);
#75778=ORIENTED_EDGE('',*,*,#53911,.T.);
#75779=ORIENTED_EDGE('',*,*,#53912,.T.);
#75780=ORIENTED_EDGE('',*,*,#53913,.F.);
#75781=ORIENTED_EDGE('',*,*,#53914,.F.);
#75782=ORIENTED_EDGE('',*,*,#53915,.F.);
#75783=ORIENTED_EDGE('',*,*,#53916,.T.);
#75784=ORIENTED_EDGE('',*,*,#53914,.T.);
#75785=ORIENTED_EDGE('',*,*,#53917,.T.);
#75786=ORIENTED_EDGE('',*,*,#53918,.T.);
#75787=ORIENTED_EDGE('',*,*,#53919,.T.);
#75788=ORIENTED_EDGE('',*,*,#52467,.F.);
#75789=ORIENTED_EDGE('',*,*,#53920,.T.);
#75790=ORIENTED_EDGE('',*,*,#53898,.F.);
#75791=ORIENTED_EDGE('',*,*,#53921,.T.);
#75792=ORIENTED_EDGE('',*,*,#53918,.F.);
#75793=ORIENTED_EDGE('',*,*,#53922,.T.);
#75794=ORIENTED_EDGE('',*,*,#52199,.F.);
#75795=ORIENTED_EDGE('',*,*,#53923,.T.);
#75796=ORIENTED_EDGE('',*,*,#53909,.F.);
#75797=ORIENTED_EDGE('',*,*,#53924,.T.);
#75798=ORIENTED_EDGE('',*,*,#53911,.F.);
#75799=ORIENTED_EDGE('',*,*,#53925,.T.);
#75800=ORIENTED_EDGE('',*,*,#53905,.F.);
#75801=ORIENTED_EDGE('',*,*,#53926,.T.);
#75802=ORIENTED_EDGE('',*,*,#53907,.F.);
#75803=ORIENTED_EDGE('',*,*,#53927,.T.);
#75804=ORIENTED_EDGE('',*,*,#53928,.T.);
#75805=ORIENTED_EDGE('',*,*,#53929,.T.);
#75806=ORIENTED_EDGE('',*,*,#53930,.F.);
#75807=ORIENTED_EDGE('',*,*,#53931,.F.);
#75808=ORIENTED_EDGE('',*,*,#53932,.F.);
#75809=ORIENTED_EDGE('',*,*,#53933,.T.);
#75810=ORIENTED_EDGE('',*,*,#53931,.T.);
#75811=ORIENTED_EDGE('',*,*,#53934,.T.);
#75812=ORIENTED_EDGE('',*,*,#53935,.T.);
#75813=ORIENTED_EDGE('',*,*,#53936,.T.);
#75814=ORIENTED_EDGE('',*,*,#53937,.T.);
#75815=ORIENTED_EDGE('',*,*,#53938,.T.);
#75816=ORIENTED_EDGE('',*,*,#53939,.T.);
#75817=ORIENTED_EDGE('',*,*,#53940,.T.);
#75818=ORIENTED_EDGE('',*,*,#53941,.T.);
#75819=ORIENTED_EDGE('',*,*,#53942,.T.);
#75820=ORIENTED_EDGE('',*,*,#53943,.F.);
#75821=ORIENTED_EDGE('',*,*,#53944,.F.);
#75822=ORIENTED_EDGE('',*,*,#53945,.F.);
#75823=ORIENTED_EDGE('',*,*,#53946,.T.);
#75824=ORIENTED_EDGE('',*,*,#53944,.T.);
#75825=ORIENTED_EDGE('',*,*,#53947,.T.);
#75826=ORIENTED_EDGE('',*,*,#53948,.T.);
#75827=ORIENTED_EDGE('',*,*,#53949,.T.);
#75828=ORIENTED_EDGE('',*,*,#52473,.F.);
#75829=ORIENTED_EDGE('',*,*,#53950,.T.);
#75830=ORIENTED_EDGE('',*,*,#53928,.F.);
#75831=ORIENTED_EDGE('',*,*,#53951,.T.);
#75832=ORIENTED_EDGE('',*,*,#53948,.F.);
#75833=ORIENTED_EDGE('',*,*,#53952,.T.);
#75834=ORIENTED_EDGE('',*,*,#52193,.F.);
#75835=ORIENTED_EDGE('',*,*,#53953,.T.);
#75836=ORIENTED_EDGE('',*,*,#53939,.F.);
#75837=ORIENTED_EDGE('',*,*,#53954,.T.);
#75838=ORIENTED_EDGE('',*,*,#53941,.F.);
#75839=ORIENTED_EDGE('',*,*,#53955,.T.);
#75840=ORIENTED_EDGE('',*,*,#53935,.F.);
#75841=ORIENTED_EDGE('',*,*,#53956,.T.);
#75842=ORIENTED_EDGE('',*,*,#53937,.F.);
#75843=ORIENTED_EDGE('',*,*,#53957,.T.);
#75844=ORIENTED_EDGE('',*,*,#53958,.T.);
#75845=ORIENTED_EDGE('',*,*,#53959,.T.);
#75846=ORIENTED_EDGE('',*,*,#53960,.F.);
#75847=ORIENTED_EDGE('',*,*,#53961,.F.);
#75848=ORIENTED_EDGE('',*,*,#53962,.F.);
#75849=ORIENTED_EDGE('',*,*,#53963,.T.);
#75850=ORIENTED_EDGE('',*,*,#53961,.T.);
#75851=ORIENTED_EDGE('',*,*,#53964,.T.);
#75852=ORIENTED_EDGE('',*,*,#53965,.T.);
#75853=ORIENTED_EDGE('',*,*,#53966,.T.);
#75854=ORIENTED_EDGE('',*,*,#53967,.T.);
#75855=ORIENTED_EDGE('',*,*,#53968,.T.);
#75856=ORIENTED_EDGE('',*,*,#53969,.T.);
#75857=ORIENTED_EDGE('',*,*,#53970,.T.);
#75858=ORIENTED_EDGE('',*,*,#53971,.T.);
#75859=ORIENTED_EDGE('',*,*,#53972,.T.);
#75860=ORIENTED_EDGE('',*,*,#53973,.F.);
#75861=ORIENTED_EDGE('',*,*,#53974,.F.);
#75862=ORIENTED_EDGE('',*,*,#53975,.F.);
#75863=ORIENTED_EDGE('',*,*,#53976,.T.);
#75864=ORIENTED_EDGE('',*,*,#53974,.T.);
#75865=ORIENTED_EDGE('',*,*,#53977,.T.);
#75866=ORIENTED_EDGE('',*,*,#53978,.T.);
#75867=ORIENTED_EDGE('',*,*,#53979,.T.);
#75868=ORIENTED_EDGE('',*,*,#52479,.F.);
#75869=ORIENTED_EDGE('',*,*,#53980,.T.);
#75870=ORIENTED_EDGE('',*,*,#53958,.F.);
#75871=ORIENTED_EDGE('',*,*,#53981,.T.);
#75872=ORIENTED_EDGE('',*,*,#53978,.F.);
#75873=ORIENTED_EDGE('',*,*,#53982,.T.);
#75874=ORIENTED_EDGE('',*,*,#52187,.F.);
#75875=ORIENTED_EDGE('',*,*,#53983,.T.);
#75876=ORIENTED_EDGE('',*,*,#53969,.F.);
#75877=ORIENTED_EDGE('',*,*,#53984,.T.);
#75878=ORIENTED_EDGE('',*,*,#53971,.F.);
#75879=ORIENTED_EDGE('',*,*,#53985,.T.);
#75880=ORIENTED_EDGE('',*,*,#53965,.F.);
#75881=ORIENTED_EDGE('',*,*,#53986,.T.);
#75882=ORIENTED_EDGE('',*,*,#53967,.F.);
#75883=ORIENTED_EDGE('',*,*,#53987,.T.);
#75884=ORIENTED_EDGE('',*,*,#53988,.T.);
#75885=ORIENTED_EDGE('',*,*,#53989,.T.);
#75886=ORIENTED_EDGE('',*,*,#53990,.F.);
#75887=ORIENTED_EDGE('',*,*,#53991,.F.);
#75888=ORIENTED_EDGE('',*,*,#53992,.F.);
#75889=ORIENTED_EDGE('',*,*,#53993,.T.);
#75890=ORIENTED_EDGE('',*,*,#53991,.T.);
#75891=ORIENTED_EDGE('',*,*,#53994,.T.);
#75892=ORIENTED_EDGE('',*,*,#53995,.T.);
#75893=ORIENTED_EDGE('',*,*,#53996,.T.);
#75894=ORIENTED_EDGE('',*,*,#53997,.T.);
#75895=ORIENTED_EDGE('',*,*,#53998,.T.);
#75896=ORIENTED_EDGE('',*,*,#53999,.T.);
#75897=ORIENTED_EDGE('',*,*,#54000,.T.);
#75898=ORIENTED_EDGE('',*,*,#54001,.T.);
#75899=ORIENTED_EDGE('',*,*,#54002,.T.);
#75900=ORIENTED_EDGE('',*,*,#54003,.F.);
#75901=ORIENTED_EDGE('',*,*,#54004,.F.);
#75902=ORIENTED_EDGE('',*,*,#54005,.F.);
#75903=ORIENTED_EDGE('',*,*,#54006,.T.);
#75904=ORIENTED_EDGE('',*,*,#54004,.T.);
#75905=ORIENTED_EDGE('',*,*,#54007,.T.);
#75906=ORIENTED_EDGE('',*,*,#54008,.T.);
#75907=ORIENTED_EDGE('',*,*,#54009,.T.);
#75908=ORIENTED_EDGE('',*,*,#52485,.F.);
#75909=ORIENTED_EDGE('',*,*,#54010,.T.);
#75910=ORIENTED_EDGE('',*,*,#53988,.F.);
#75911=ORIENTED_EDGE('',*,*,#54011,.T.);
#75912=ORIENTED_EDGE('',*,*,#54008,.F.);
#75913=ORIENTED_EDGE('',*,*,#54012,.T.);
#75914=ORIENTED_EDGE('',*,*,#52181,.F.);
#75915=ORIENTED_EDGE('',*,*,#54013,.T.);
#75916=ORIENTED_EDGE('',*,*,#53999,.F.);
#75917=ORIENTED_EDGE('',*,*,#54014,.T.);
#75918=ORIENTED_EDGE('',*,*,#54001,.F.);
#75919=ORIENTED_EDGE('',*,*,#54015,.T.);
#75920=ORIENTED_EDGE('',*,*,#53995,.F.);
#75921=ORIENTED_EDGE('',*,*,#54016,.T.);
#75922=ORIENTED_EDGE('',*,*,#53997,.F.);
#75923=ORIENTED_EDGE('',*,*,#54017,.T.);
#75924=ORIENTED_EDGE('',*,*,#54018,.T.);
#75925=ORIENTED_EDGE('',*,*,#54019,.T.);
#75926=ORIENTED_EDGE('',*,*,#54020,.F.);
#75927=ORIENTED_EDGE('',*,*,#54021,.F.);
#75928=ORIENTED_EDGE('',*,*,#54022,.F.);
#75929=ORIENTED_EDGE('',*,*,#54023,.T.);
#75930=ORIENTED_EDGE('',*,*,#54021,.T.);
#75931=ORIENTED_EDGE('',*,*,#54024,.T.);
#75932=ORIENTED_EDGE('',*,*,#54025,.T.);
#75933=ORIENTED_EDGE('',*,*,#54026,.T.);
#75934=ORIENTED_EDGE('',*,*,#54027,.T.);
#75935=ORIENTED_EDGE('',*,*,#54028,.T.);
#75936=ORIENTED_EDGE('',*,*,#54029,.T.);
#75937=ORIENTED_EDGE('',*,*,#54030,.T.);
#75938=ORIENTED_EDGE('',*,*,#54031,.T.);
#75939=ORIENTED_EDGE('',*,*,#54032,.T.);
#75940=ORIENTED_EDGE('',*,*,#54033,.F.);
#75941=ORIENTED_EDGE('',*,*,#54034,.F.);
#75942=ORIENTED_EDGE('',*,*,#54035,.F.);
#75943=ORIENTED_EDGE('',*,*,#54036,.T.);
#75944=ORIENTED_EDGE('',*,*,#54034,.T.);
#75945=ORIENTED_EDGE('',*,*,#54037,.T.);
#75946=ORIENTED_EDGE('',*,*,#54038,.T.);
#75947=ORIENTED_EDGE('',*,*,#54039,.T.);
#75948=ORIENTED_EDGE('',*,*,#52491,.F.);
#75949=ORIENTED_EDGE('',*,*,#54040,.T.);
#75950=ORIENTED_EDGE('',*,*,#54018,.F.);
#75951=ORIENTED_EDGE('',*,*,#54041,.T.);
#75952=ORIENTED_EDGE('',*,*,#54038,.F.);
#75953=ORIENTED_EDGE('',*,*,#54042,.T.);
#75954=ORIENTED_EDGE('',*,*,#52175,.F.);
#75955=ORIENTED_EDGE('',*,*,#54043,.T.);
#75956=ORIENTED_EDGE('',*,*,#54029,.F.);
#75957=ORIENTED_EDGE('',*,*,#54044,.T.);
#75958=ORIENTED_EDGE('',*,*,#54031,.F.);
#75959=ORIENTED_EDGE('',*,*,#54045,.T.);
#75960=ORIENTED_EDGE('',*,*,#54025,.F.);
#75961=ORIENTED_EDGE('',*,*,#54046,.T.);
#75962=ORIENTED_EDGE('',*,*,#54027,.F.);
#75963=ORIENTED_EDGE('',*,*,#54047,.T.);
#75964=ORIENTED_EDGE('',*,*,#54048,.T.);
#75965=ORIENTED_EDGE('',*,*,#54049,.T.);
#75966=ORIENTED_EDGE('',*,*,#54050,.F.);
#75967=ORIENTED_EDGE('',*,*,#54051,.F.);
#75968=ORIENTED_EDGE('',*,*,#54052,.F.);
#75969=ORIENTED_EDGE('',*,*,#54053,.T.);
#75970=ORIENTED_EDGE('',*,*,#54051,.T.);
#75971=ORIENTED_EDGE('',*,*,#54054,.T.);
#75972=ORIENTED_EDGE('',*,*,#54055,.T.);
#75973=ORIENTED_EDGE('',*,*,#54056,.T.);
#75974=ORIENTED_EDGE('',*,*,#54057,.T.);
#75975=ORIENTED_EDGE('',*,*,#54058,.T.);
#75976=ORIENTED_EDGE('',*,*,#54059,.T.);
#75977=ORIENTED_EDGE('',*,*,#54060,.T.);
#75978=ORIENTED_EDGE('',*,*,#54061,.T.);
#75979=ORIENTED_EDGE('',*,*,#54062,.T.);
#75980=ORIENTED_EDGE('',*,*,#54063,.F.);
#75981=ORIENTED_EDGE('',*,*,#54064,.F.);
#75982=ORIENTED_EDGE('',*,*,#54065,.F.);
#75983=ORIENTED_EDGE('',*,*,#54066,.T.);
#75984=ORIENTED_EDGE('',*,*,#54064,.T.);
#75985=ORIENTED_EDGE('',*,*,#54067,.T.);
#75986=ORIENTED_EDGE('',*,*,#54068,.T.);
#75987=ORIENTED_EDGE('',*,*,#54069,.T.);
#75988=ORIENTED_EDGE('',*,*,#52497,.F.);
#75989=ORIENTED_EDGE('',*,*,#54070,.T.);
#75990=ORIENTED_EDGE('',*,*,#54048,.F.);
#75991=ORIENTED_EDGE('',*,*,#54071,.T.);
#75992=ORIENTED_EDGE('',*,*,#54068,.F.);
#75993=ORIENTED_EDGE('',*,*,#54072,.T.);
#75994=ORIENTED_EDGE('',*,*,#52169,.F.);
#75995=ORIENTED_EDGE('',*,*,#54073,.T.);
#75996=ORIENTED_EDGE('',*,*,#54059,.F.);
#75997=ORIENTED_EDGE('',*,*,#54074,.T.);
#75998=ORIENTED_EDGE('',*,*,#54061,.F.);
#75999=ORIENTED_EDGE('',*,*,#54075,.T.);
#76000=ORIENTED_EDGE('',*,*,#54055,.F.);
#76001=ORIENTED_EDGE('',*,*,#54076,.T.);
#76002=ORIENTED_EDGE('',*,*,#54057,.F.);
#76003=ORIENTED_EDGE('',*,*,#54077,.T.);
#76004=ORIENTED_EDGE('',*,*,#54078,.T.);
#76005=ORIENTED_EDGE('',*,*,#54079,.T.);
#76006=ORIENTED_EDGE('',*,*,#54080,.F.);
#76007=ORIENTED_EDGE('',*,*,#54081,.F.);
#76008=ORIENTED_EDGE('',*,*,#54082,.F.);
#76009=ORIENTED_EDGE('',*,*,#54083,.T.);
#76010=ORIENTED_EDGE('',*,*,#54081,.T.);
#76011=ORIENTED_EDGE('',*,*,#54084,.T.);
#76012=ORIENTED_EDGE('',*,*,#54085,.T.);
#76013=ORIENTED_EDGE('',*,*,#54086,.T.);
#76014=ORIENTED_EDGE('',*,*,#54087,.T.);
#76015=ORIENTED_EDGE('',*,*,#54088,.T.);
#76016=ORIENTED_EDGE('',*,*,#54089,.T.);
#76017=ORIENTED_EDGE('',*,*,#54090,.T.);
#76018=ORIENTED_EDGE('',*,*,#54091,.T.);
#76019=ORIENTED_EDGE('',*,*,#54092,.T.);
#76020=ORIENTED_EDGE('',*,*,#54093,.F.);
#76021=ORIENTED_EDGE('',*,*,#54094,.F.);
#76022=ORIENTED_EDGE('',*,*,#54095,.F.);
#76023=ORIENTED_EDGE('',*,*,#54096,.T.);
#76024=ORIENTED_EDGE('',*,*,#54094,.T.);
#76025=ORIENTED_EDGE('',*,*,#54097,.T.);
#76026=ORIENTED_EDGE('',*,*,#54098,.T.);
#76027=ORIENTED_EDGE('',*,*,#54099,.T.);
#76028=ORIENTED_EDGE('',*,*,#52503,.F.);
#76029=ORIENTED_EDGE('',*,*,#54100,.T.);
#76030=ORIENTED_EDGE('',*,*,#54078,.F.);
#76031=ORIENTED_EDGE('',*,*,#54101,.T.);
#76032=ORIENTED_EDGE('',*,*,#54098,.F.);
#76033=ORIENTED_EDGE('',*,*,#54102,.T.);
#76034=ORIENTED_EDGE('',*,*,#52163,.F.);
#76035=ORIENTED_EDGE('',*,*,#54103,.T.);
#76036=ORIENTED_EDGE('',*,*,#54089,.F.);
#76037=ORIENTED_EDGE('',*,*,#54104,.T.);
#76038=ORIENTED_EDGE('',*,*,#54091,.F.);
#76039=ORIENTED_EDGE('',*,*,#54105,.T.);
#76040=ORIENTED_EDGE('',*,*,#54085,.F.);
#76041=ORIENTED_EDGE('',*,*,#54106,.T.);
#76042=ORIENTED_EDGE('',*,*,#54087,.F.);
#76043=ORIENTED_EDGE('',*,*,#54107,.T.);
#76044=ORIENTED_EDGE('',*,*,#54108,.T.);
#76045=ORIENTED_EDGE('',*,*,#54109,.T.);
#76046=ORIENTED_EDGE('',*,*,#54110,.F.);
#76047=ORIENTED_EDGE('',*,*,#54111,.F.);
#76048=ORIENTED_EDGE('',*,*,#54112,.F.);
#76049=ORIENTED_EDGE('',*,*,#54113,.T.);
#76050=ORIENTED_EDGE('',*,*,#54111,.T.);
#76051=ORIENTED_EDGE('',*,*,#54114,.T.);
#76052=ORIENTED_EDGE('',*,*,#54115,.T.);
#76053=ORIENTED_EDGE('',*,*,#54116,.T.);
#76054=ORIENTED_EDGE('',*,*,#54117,.T.);
#76055=ORIENTED_EDGE('',*,*,#54118,.T.);
#76056=ORIENTED_EDGE('',*,*,#54119,.T.);
#76057=ORIENTED_EDGE('',*,*,#54120,.T.);
#76058=ORIENTED_EDGE('',*,*,#54121,.T.);
#76059=ORIENTED_EDGE('',*,*,#54122,.T.);
#76060=ORIENTED_EDGE('',*,*,#54123,.F.);
#76061=ORIENTED_EDGE('',*,*,#54124,.F.);
#76062=ORIENTED_EDGE('',*,*,#54125,.F.);
#76063=ORIENTED_EDGE('',*,*,#54126,.T.);
#76064=ORIENTED_EDGE('',*,*,#54124,.T.);
#76065=ORIENTED_EDGE('',*,*,#54127,.T.);
#76066=ORIENTED_EDGE('',*,*,#54128,.T.);
#76067=ORIENTED_EDGE('',*,*,#54129,.T.);
#76068=ORIENTED_EDGE('',*,*,#52509,.F.);
#76069=ORIENTED_EDGE('',*,*,#54130,.T.);
#76070=ORIENTED_EDGE('',*,*,#54108,.F.);
#76071=ORIENTED_EDGE('',*,*,#54131,.T.);
#76072=ORIENTED_EDGE('',*,*,#54128,.F.);
#76073=ORIENTED_EDGE('',*,*,#54132,.T.);
#76074=ORIENTED_EDGE('',*,*,#52157,.F.);
#76075=ORIENTED_EDGE('',*,*,#54133,.T.);
#76076=ORIENTED_EDGE('',*,*,#54119,.F.);
#76077=ORIENTED_EDGE('',*,*,#54134,.T.);
#76078=ORIENTED_EDGE('',*,*,#54121,.F.);
#76079=ORIENTED_EDGE('',*,*,#54135,.T.);
#76080=ORIENTED_EDGE('',*,*,#54115,.F.);
#76081=ORIENTED_EDGE('',*,*,#54136,.T.);
#76082=ORIENTED_EDGE('',*,*,#54117,.F.);
#76083=ORIENTED_EDGE('',*,*,#54137,.T.);
#76084=ORIENTED_EDGE('',*,*,#54138,.T.);
#76085=ORIENTED_EDGE('',*,*,#54139,.T.);
#76086=ORIENTED_EDGE('',*,*,#54140,.F.);
#76087=ORIENTED_EDGE('',*,*,#54141,.F.);
#76088=ORIENTED_EDGE('',*,*,#54142,.F.);
#76089=ORIENTED_EDGE('',*,*,#54143,.T.);
#76090=ORIENTED_EDGE('',*,*,#54141,.T.);
#76091=ORIENTED_EDGE('',*,*,#54144,.T.);
#76092=ORIENTED_EDGE('',*,*,#54145,.T.);
#76093=ORIENTED_EDGE('',*,*,#54146,.T.);
#76094=ORIENTED_EDGE('',*,*,#54147,.T.);
#76095=ORIENTED_EDGE('',*,*,#54148,.T.);
#76096=ORIENTED_EDGE('',*,*,#54149,.T.);
#76097=ORIENTED_EDGE('',*,*,#54150,.T.);
#76098=ORIENTED_EDGE('',*,*,#54151,.T.);
#76099=ORIENTED_EDGE('',*,*,#54152,.T.);
#76100=ORIENTED_EDGE('',*,*,#54153,.F.);
#76101=ORIENTED_EDGE('',*,*,#54154,.F.);
#76102=ORIENTED_EDGE('',*,*,#54155,.F.);
#76103=ORIENTED_EDGE('',*,*,#54156,.T.);
#76104=ORIENTED_EDGE('',*,*,#54154,.T.);
#76105=ORIENTED_EDGE('',*,*,#54157,.T.);
#76106=ORIENTED_EDGE('',*,*,#54158,.T.);
#76107=ORIENTED_EDGE('',*,*,#54159,.T.);
#76108=ORIENTED_EDGE('',*,*,#52515,.F.);
#76109=ORIENTED_EDGE('',*,*,#54160,.T.);
#76110=ORIENTED_EDGE('',*,*,#54138,.F.);
#76111=ORIENTED_EDGE('',*,*,#54161,.T.);
#76112=ORIENTED_EDGE('',*,*,#54158,.F.);
#76113=ORIENTED_EDGE('',*,*,#54162,.T.);
#76114=ORIENTED_EDGE('',*,*,#52151,.F.);
#76115=ORIENTED_EDGE('',*,*,#54163,.T.);
#76116=ORIENTED_EDGE('',*,*,#54149,.F.);
#76117=ORIENTED_EDGE('',*,*,#54164,.T.);
#76118=ORIENTED_EDGE('',*,*,#54151,.F.);
#76119=ORIENTED_EDGE('',*,*,#54165,.T.);
#76120=ORIENTED_EDGE('',*,*,#54145,.F.);
#76121=ORIENTED_EDGE('',*,*,#54166,.T.);
#76122=ORIENTED_EDGE('',*,*,#54147,.F.);
#76123=ORIENTED_EDGE('',*,*,#54167,.T.);
#76124=ORIENTED_EDGE('',*,*,#54168,.T.);
#76125=ORIENTED_EDGE('',*,*,#54169,.T.);
#76126=ORIENTED_EDGE('',*,*,#54170,.F.);
#76127=ORIENTED_EDGE('',*,*,#54171,.F.);
#76128=ORIENTED_EDGE('',*,*,#54172,.F.);
#76129=ORIENTED_EDGE('',*,*,#54173,.T.);
#76130=ORIENTED_EDGE('',*,*,#54171,.T.);
#76131=ORIENTED_EDGE('',*,*,#54174,.T.);
#76132=ORIENTED_EDGE('',*,*,#54175,.T.);
#76133=ORIENTED_EDGE('',*,*,#54176,.T.);
#76134=ORIENTED_EDGE('',*,*,#54177,.T.);
#76135=ORIENTED_EDGE('',*,*,#54178,.T.);
#76136=ORIENTED_EDGE('',*,*,#54179,.T.);
#76137=ORIENTED_EDGE('',*,*,#54180,.T.);
#76138=ORIENTED_EDGE('',*,*,#54181,.T.);
#76139=ORIENTED_EDGE('',*,*,#54182,.T.);
#76140=ORIENTED_EDGE('',*,*,#54183,.F.);
#76141=ORIENTED_EDGE('',*,*,#54184,.F.);
#76142=ORIENTED_EDGE('',*,*,#54185,.F.);
#76143=ORIENTED_EDGE('',*,*,#54186,.T.);
#76144=ORIENTED_EDGE('',*,*,#54184,.T.);
#76145=ORIENTED_EDGE('',*,*,#54187,.T.);
#76146=ORIENTED_EDGE('',*,*,#54188,.T.);
#76147=ORIENTED_EDGE('',*,*,#54189,.T.);
#76148=ORIENTED_EDGE('',*,*,#52521,.F.);
#76149=ORIENTED_EDGE('',*,*,#54190,.T.);
#76150=ORIENTED_EDGE('',*,*,#54168,.F.);
#76151=ORIENTED_EDGE('',*,*,#54191,.T.);
#76152=ORIENTED_EDGE('',*,*,#54188,.F.);
#76153=ORIENTED_EDGE('',*,*,#54192,.T.);
#76154=ORIENTED_EDGE('',*,*,#52145,.F.);
#76155=ORIENTED_EDGE('',*,*,#54193,.T.);
#76156=ORIENTED_EDGE('',*,*,#54179,.F.);
#76157=ORIENTED_EDGE('',*,*,#54194,.T.);
#76158=ORIENTED_EDGE('',*,*,#54181,.F.);
#76159=ORIENTED_EDGE('',*,*,#54195,.T.);
#76160=ORIENTED_EDGE('',*,*,#54175,.F.);
#76161=ORIENTED_EDGE('',*,*,#54196,.T.);
#76162=ORIENTED_EDGE('',*,*,#54177,.F.);
#76163=ORIENTED_EDGE('',*,*,#54197,.T.);
#76164=ORIENTED_EDGE('',*,*,#54198,.T.);
#76165=ORIENTED_EDGE('',*,*,#54199,.T.);
#76166=ORIENTED_EDGE('',*,*,#54200,.F.);
#76167=ORIENTED_EDGE('',*,*,#54201,.F.);
#76168=ORIENTED_EDGE('',*,*,#54202,.F.);
#76169=ORIENTED_EDGE('',*,*,#54203,.T.);
#76170=ORIENTED_EDGE('',*,*,#54201,.T.);
#76171=ORIENTED_EDGE('',*,*,#54204,.T.);
#76172=ORIENTED_EDGE('',*,*,#54205,.T.);
#76173=ORIENTED_EDGE('',*,*,#54206,.T.);
#76174=ORIENTED_EDGE('',*,*,#54207,.T.);
#76175=ORIENTED_EDGE('',*,*,#54208,.T.);
#76176=ORIENTED_EDGE('',*,*,#54209,.T.);
#76177=ORIENTED_EDGE('',*,*,#54210,.T.);
#76178=ORIENTED_EDGE('',*,*,#54211,.T.);
#76179=ORIENTED_EDGE('',*,*,#54212,.T.);
#76180=ORIENTED_EDGE('',*,*,#54213,.F.);
#76181=ORIENTED_EDGE('',*,*,#54214,.F.);
#76182=ORIENTED_EDGE('',*,*,#54215,.F.);
#76183=ORIENTED_EDGE('',*,*,#54216,.T.);
#76184=ORIENTED_EDGE('',*,*,#54214,.T.);
#76185=ORIENTED_EDGE('',*,*,#54217,.T.);
#76186=ORIENTED_EDGE('',*,*,#54218,.T.);
#76187=ORIENTED_EDGE('',*,*,#54219,.T.);
#76188=ORIENTED_EDGE('',*,*,#52527,.F.);
#76189=ORIENTED_EDGE('',*,*,#54220,.T.);
#76190=ORIENTED_EDGE('',*,*,#54198,.F.);
#76191=ORIENTED_EDGE('',*,*,#54221,.T.);
#76192=ORIENTED_EDGE('',*,*,#54218,.F.);
#76193=ORIENTED_EDGE('',*,*,#54222,.T.);
#76194=ORIENTED_EDGE('',*,*,#52139,.F.);
#76195=ORIENTED_EDGE('',*,*,#54223,.T.);
#76196=ORIENTED_EDGE('',*,*,#54209,.F.);
#76197=ORIENTED_EDGE('',*,*,#54224,.T.);
#76198=ORIENTED_EDGE('',*,*,#54211,.F.);
#76199=ORIENTED_EDGE('',*,*,#54225,.T.);
#76200=ORIENTED_EDGE('',*,*,#54205,.F.);
#76201=ORIENTED_EDGE('',*,*,#54226,.T.);
#76202=ORIENTED_EDGE('',*,*,#54207,.F.);
#76203=ORIENTED_EDGE('',*,*,#54227,.T.);
#76204=ORIENTED_EDGE('',*,*,#54228,.T.);
#76205=ORIENTED_EDGE('',*,*,#54229,.T.);
#76206=ORIENTED_EDGE('',*,*,#54230,.F.);
#76207=ORIENTED_EDGE('',*,*,#54231,.F.);
#76208=ORIENTED_EDGE('',*,*,#54232,.F.);
#76209=ORIENTED_EDGE('',*,*,#54233,.T.);
#76210=ORIENTED_EDGE('',*,*,#54231,.T.);
#76211=ORIENTED_EDGE('',*,*,#54234,.T.);
#76212=ORIENTED_EDGE('',*,*,#54235,.T.);
#76213=ORIENTED_EDGE('',*,*,#54236,.T.);
#76214=ORIENTED_EDGE('',*,*,#54237,.T.);
#76215=ORIENTED_EDGE('',*,*,#54238,.T.);
#76216=ORIENTED_EDGE('',*,*,#54239,.T.);
#76217=ORIENTED_EDGE('',*,*,#54240,.T.);
#76218=ORIENTED_EDGE('',*,*,#54241,.T.);
#76219=ORIENTED_EDGE('',*,*,#54242,.T.);
#76220=ORIENTED_EDGE('',*,*,#54243,.F.);
#76221=ORIENTED_EDGE('',*,*,#54244,.F.);
#76222=ORIENTED_EDGE('',*,*,#54245,.F.);
#76223=ORIENTED_EDGE('',*,*,#54246,.T.);
#76224=ORIENTED_EDGE('',*,*,#54244,.T.);
#76225=ORIENTED_EDGE('',*,*,#54247,.T.);
#76226=ORIENTED_EDGE('',*,*,#54248,.T.);
#76227=ORIENTED_EDGE('',*,*,#54249,.T.);
#76228=ORIENTED_EDGE('',*,*,#52533,.F.);
#76229=ORIENTED_EDGE('',*,*,#54250,.T.);
#76230=ORIENTED_EDGE('',*,*,#54228,.F.);
#76231=ORIENTED_EDGE('',*,*,#54251,.T.);
#76232=ORIENTED_EDGE('',*,*,#54248,.F.);
#76233=ORIENTED_EDGE('',*,*,#54252,.T.);
#76234=ORIENTED_EDGE('',*,*,#52133,.F.);
#76235=ORIENTED_EDGE('',*,*,#54253,.T.);
#76236=ORIENTED_EDGE('',*,*,#54239,.F.);
#76237=ORIENTED_EDGE('',*,*,#54254,.T.);
#76238=ORIENTED_EDGE('',*,*,#54241,.F.);
#76239=ORIENTED_EDGE('',*,*,#54255,.T.);
#76240=ORIENTED_EDGE('',*,*,#54235,.F.);
#76241=ORIENTED_EDGE('',*,*,#54256,.T.);
#76242=ORIENTED_EDGE('',*,*,#54237,.F.);
#76243=ORIENTED_EDGE('',*,*,#54257,.T.);
#76244=ORIENTED_EDGE('',*,*,#54258,.T.);
#76245=ORIENTED_EDGE('',*,*,#54259,.T.);
#76246=ORIENTED_EDGE('',*,*,#54260,.F.);
#76247=ORIENTED_EDGE('',*,*,#54261,.F.);
#76248=ORIENTED_EDGE('',*,*,#54262,.F.);
#76249=ORIENTED_EDGE('',*,*,#54263,.T.);
#76250=ORIENTED_EDGE('',*,*,#54261,.T.);
#76251=ORIENTED_EDGE('',*,*,#54264,.T.);
#76252=ORIENTED_EDGE('',*,*,#54265,.T.);
#76253=ORIENTED_EDGE('',*,*,#54266,.T.);
#76254=ORIENTED_EDGE('',*,*,#54267,.T.);
#76255=ORIENTED_EDGE('',*,*,#54268,.T.);
#76256=ORIENTED_EDGE('',*,*,#54269,.T.);
#76257=ORIENTED_EDGE('',*,*,#54270,.T.);
#76258=ORIENTED_EDGE('',*,*,#54271,.T.);
#76259=ORIENTED_EDGE('',*,*,#54272,.T.);
#76260=ORIENTED_EDGE('',*,*,#54273,.F.);
#76261=ORIENTED_EDGE('',*,*,#54274,.F.);
#76262=ORIENTED_EDGE('',*,*,#54275,.F.);
#76263=ORIENTED_EDGE('',*,*,#54276,.T.);
#76264=ORIENTED_EDGE('',*,*,#54274,.T.);
#76265=ORIENTED_EDGE('',*,*,#54277,.T.);
#76266=ORIENTED_EDGE('',*,*,#54278,.T.);
#76267=ORIENTED_EDGE('',*,*,#54279,.T.);
#76268=ORIENTED_EDGE('',*,*,#52539,.F.);
#76269=ORIENTED_EDGE('',*,*,#54280,.T.);
#76270=ORIENTED_EDGE('',*,*,#54258,.F.);
#76271=ORIENTED_EDGE('',*,*,#54281,.T.);
#76272=ORIENTED_EDGE('',*,*,#54278,.F.);
#76273=ORIENTED_EDGE('',*,*,#54282,.T.);
#76274=ORIENTED_EDGE('',*,*,#52127,.F.);
#76275=ORIENTED_EDGE('',*,*,#54283,.T.);
#76276=ORIENTED_EDGE('',*,*,#54269,.F.);
#76277=ORIENTED_EDGE('',*,*,#54284,.T.);
#76278=ORIENTED_EDGE('',*,*,#54271,.F.);
#76279=ORIENTED_EDGE('',*,*,#54285,.T.);
#76280=ORIENTED_EDGE('',*,*,#54265,.F.);
#76281=ORIENTED_EDGE('',*,*,#54286,.T.);
#76282=ORIENTED_EDGE('',*,*,#54267,.F.);
#76283=ORIENTED_EDGE('',*,*,#54287,.T.);
#76284=ORIENTED_EDGE('',*,*,#54288,.T.);
#76285=ORIENTED_EDGE('',*,*,#54289,.T.);
#76286=ORIENTED_EDGE('',*,*,#54290,.F.);
#76287=ORIENTED_EDGE('',*,*,#54291,.F.);
#76288=ORIENTED_EDGE('',*,*,#54292,.F.);
#76289=ORIENTED_EDGE('',*,*,#54293,.T.);
#76290=ORIENTED_EDGE('',*,*,#54291,.T.);
#76291=ORIENTED_EDGE('',*,*,#54294,.T.);
#76292=ORIENTED_EDGE('',*,*,#54295,.T.);
#76293=ORIENTED_EDGE('',*,*,#54296,.T.);
#76294=ORIENTED_EDGE('',*,*,#54297,.T.);
#76295=ORIENTED_EDGE('',*,*,#54298,.T.);
#76296=ORIENTED_EDGE('',*,*,#54299,.T.);
#76297=ORIENTED_EDGE('',*,*,#54300,.T.);
#76298=ORIENTED_EDGE('',*,*,#54301,.T.);
#76299=ORIENTED_EDGE('',*,*,#54302,.T.);
#76300=ORIENTED_EDGE('',*,*,#54303,.F.);
#76301=ORIENTED_EDGE('',*,*,#54304,.F.);
#76302=ORIENTED_EDGE('',*,*,#54305,.F.);
#76303=ORIENTED_EDGE('',*,*,#54306,.T.);
#76304=ORIENTED_EDGE('',*,*,#54304,.T.);
#76305=ORIENTED_EDGE('',*,*,#54307,.T.);
#76306=ORIENTED_EDGE('',*,*,#54308,.T.);
#76307=ORIENTED_EDGE('',*,*,#54309,.T.);
#76308=ORIENTED_EDGE('',*,*,#52545,.F.);
#76309=ORIENTED_EDGE('',*,*,#54310,.T.);
#76310=ORIENTED_EDGE('',*,*,#54288,.F.);
#76311=ORIENTED_EDGE('',*,*,#54311,.T.);
#76312=ORIENTED_EDGE('',*,*,#54308,.F.);
#76313=ORIENTED_EDGE('',*,*,#54312,.T.);
#76314=ORIENTED_EDGE('',*,*,#52121,.F.);
#76315=ORIENTED_EDGE('',*,*,#54313,.T.);
#76316=ORIENTED_EDGE('',*,*,#54299,.F.);
#76317=ORIENTED_EDGE('',*,*,#54314,.T.);
#76318=ORIENTED_EDGE('',*,*,#54301,.F.);
#76319=ORIENTED_EDGE('',*,*,#54315,.T.);
#76320=ORIENTED_EDGE('',*,*,#54295,.F.);
#76321=ORIENTED_EDGE('',*,*,#54316,.T.);
#76322=ORIENTED_EDGE('',*,*,#54297,.F.);
#76323=ORIENTED_EDGE('',*,*,#54317,.T.);
#76324=ORIENTED_EDGE('',*,*,#54318,.T.);
#76325=ORIENTED_EDGE('',*,*,#54319,.T.);
#76326=ORIENTED_EDGE('',*,*,#54320,.F.);
#76327=ORIENTED_EDGE('',*,*,#54321,.F.);
#76328=ORIENTED_EDGE('',*,*,#54322,.F.);
#76329=ORIENTED_EDGE('',*,*,#54323,.T.);
#76330=ORIENTED_EDGE('',*,*,#54321,.T.);
#76331=ORIENTED_EDGE('',*,*,#54324,.T.);
#76332=ORIENTED_EDGE('',*,*,#54325,.T.);
#76333=ORIENTED_EDGE('',*,*,#54326,.T.);
#76334=ORIENTED_EDGE('',*,*,#54327,.T.);
#76335=ORIENTED_EDGE('',*,*,#54328,.T.);
#76336=ORIENTED_EDGE('',*,*,#54329,.T.);
#76337=ORIENTED_EDGE('',*,*,#54330,.T.);
#76338=ORIENTED_EDGE('',*,*,#54331,.T.);
#76339=ORIENTED_EDGE('',*,*,#54332,.T.);
#76340=ORIENTED_EDGE('',*,*,#54333,.F.);
#76341=ORIENTED_EDGE('',*,*,#54334,.F.);
#76342=ORIENTED_EDGE('',*,*,#54335,.F.);
#76343=ORIENTED_EDGE('',*,*,#54336,.T.);
#76344=ORIENTED_EDGE('',*,*,#54334,.T.);
#76345=ORIENTED_EDGE('',*,*,#54337,.T.);
#76346=ORIENTED_EDGE('',*,*,#54338,.T.);
#76347=ORIENTED_EDGE('',*,*,#54339,.T.);
#76348=ORIENTED_EDGE('',*,*,#52551,.F.);
#76349=ORIENTED_EDGE('',*,*,#54340,.T.);
#76350=ORIENTED_EDGE('',*,*,#54318,.F.);
#76351=ORIENTED_EDGE('',*,*,#54341,.T.);
#76352=ORIENTED_EDGE('',*,*,#54338,.F.);
#76353=ORIENTED_EDGE('',*,*,#54342,.T.);
#76354=ORIENTED_EDGE('',*,*,#52115,.F.);
#76355=ORIENTED_EDGE('',*,*,#54343,.T.);
#76356=ORIENTED_EDGE('',*,*,#54329,.F.);
#76357=ORIENTED_EDGE('',*,*,#54344,.T.);
#76358=ORIENTED_EDGE('',*,*,#54331,.F.);
#76359=ORIENTED_EDGE('',*,*,#54345,.T.);
#76360=ORIENTED_EDGE('',*,*,#54325,.F.);
#76361=ORIENTED_EDGE('',*,*,#54346,.T.);
#76362=ORIENTED_EDGE('',*,*,#54327,.F.);
#76363=ORIENTED_EDGE('',*,*,#54347,.T.);
#76364=ORIENTED_EDGE('',*,*,#54348,.T.);
#76365=ORIENTED_EDGE('',*,*,#54349,.T.);
#76366=ORIENTED_EDGE('',*,*,#54350,.F.);
#76367=ORIENTED_EDGE('',*,*,#54351,.F.);
#76368=ORIENTED_EDGE('',*,*,#54352,.F.);
#76369=ORIENTED_EDGE('',*,*,#54353,.T.);
#76370=ORIENTED_EDGE('',*,*,#54351,.T.);
#76371=ORIENTED_EDGE('',*,*,#54354,.T.);
#76372=ORIENTED_EDGE('',*,*,#54355,.T.);
#76373=ORIENTED_EDGE('',*,*,#54356,.T.);
#76374=ORIENTED_EDGE('',*,*,#54357,.T.);
#76375=ORIENTED_EDGE('',*,*,#54358,.T.);
#76376=ORIENTED_EDGE('',*,*,#54359,.T.);
#76377=ORIENTED_EDGE('',*,*,#54360,.T.);
#76378=ORIENTED_EDGE('',*,*,#54361,.T.);
#76379=ORIENTED_EDGE('',*,*,#54362,.T.);
#76380=ORIENTED_EDGE('',*,*,#54363,.F.);
#76381=ORIENTED_EDGE('',*,*,#54364,.F.);
#76382=ORIENTED_EDGE('',*,*,#54365,.F.);
#76383=ORIENTED_EDGE('',*,*,#54366,.T.);
#76384=ORIENTED_EDGE('',*,*,#54364,.T.);
#76385=ORIENTED_EDGE('',*,*,#54367,.T.);
#76386=ORIENTED_EDGE('',*,*,#54368,.T.);
#76387=ORIENTED_EDGE('',*,*,#54369,.T.);
#76388=ORIENTED_EDGE('',*,*,#52557,.F.);
#76389=ORIENTED_EDGE('',*,*,#54370,.T.);
#76390=ORIENTED_EDGE('',*,*,#54348,.F.);
#76391=ORIENTED_EDGE('',*,*,#54371,.T.);
#76392=ORIENTED_EDGE('',*,*,#54368,.F.);
#76393=ORIENTED_EDGE('',*,*,#54372,.T.);
#76394=ORIENTED_EDGE('',*,*,#52109,.F.);
#76395=ORIENTED_EDGE('',*,*,#54373,.T.);
#76396=ORIENTED_EDGE('',*,*,#54359,.F.);
#76397=ORIENTED_EDGE('',*,*,#54374,.T.);
#76398=ORIENTED_EDGE('',*,*,#54361,.F.);
#76399=ORIENTED_EDGE('',*,*,#54375,.T.);
#76400=ORIENTED_EDGE('',*,*,#54355,.F.);
#76401=ORIENTED_EDGE('',*,*,#54376,.T.);
#76402=ORIENTED_EDGE('',*,*,#54357,.F.);
#76403=ORIENTED_EDGE('',*,*,#54377,.T.);
#76404=ORIENTED_EDGE('',*,*,#54378,.T.);
#76405=ORIENTED_EDGE('',*,*,#54379,.T.);
#76406=ORIENTED_EDGE('',*,*,#54380,.F.);
#76407=ORIENTED_EDGE('',*,*,#54381,.F.);
#76408=ORIENTED_EDGE('',*,*,#54382,.F.);
#76409=ORIENTED_EDGE('',*,*,#54383,.T.);
#76410=ORIENTED_EDGE('',*,*,#54381,.T.);
#76411=ORIENTED_EDGE('',*,*,#54384,.T.);
#76412=ORIENTED_EDGE('',*,*,#54385,.T.);
#76413=ORIENTED_EDGE('',*,*,#54386,.T.);
#76414=ORIENTED_EDGE('',*,*,#54387,.T.);
#76415=ORIENTED_EDGE('',*,*,#54388,.T.);
#76416=ORIENTED_EDGE('',*,*,#54389,.T.);
#76417=ORIENTED_EDGE('',*,*,#54390,.T.);
#76418=ORIENTED_EDGE('',*,*,#54391,.T.);
#76419=ORIENTED_EDGE('',*,*,#54392,.T.);
#76420=ORIENTED_EDGE('',*,*,#54393,.F.);
#76421=ORIENTED_EDGE('',*,*,#54394,.F.);
#76422=ORIENTED_EDGE('',*,*,#54395,.F.);
#76423=ORIENTED_EDGE('',*,*,#54396,.T.);
#76424=ORIENTED_EDGE('',*,*,#54394,.T.);
#76425=ORIENTED_EDGE('',*,*,#54397,.T.);
#76426=ORIENTED_EDGE('',*,*,#54398,.T.);
#76427=ORIENTED_EDGE('',*,*,#54399,.T.);
#76428=ORIENTED_EDGE('',*,*,#52563,.F.);
#76429=ORIENTED_EDGE('',*,*,#54400,.T.);
#76430=ORIENTED_EDGE('',*,*,#54378,.F.);
#76431=ORIENTED_EDGE('',*,*,#54401,.T.);
#76432=ORIENTED_EDGE('',*,*,#54398,.F.);
#76433=ORIENTED_EDGE('',*,*,#54402,.T.);
#76434=ORIENTED_EDGE('',*,*,#52103,.F.);
#76435=ORIENTED_EDGE('',*,*,#54403,.T.);
#76436=ORIENTED_EDGE('',*,*,#54389,.F.);
#76437=ORIENTED_EDGE('',*,*,#54404,.T.);
#76438=ORIENTED_EDGE('',*,*,#54391,.F.);
#76439=ORIENTED_EDGE('',*,*,#54405,.T.);
#76440=ORIENTED_EDGE('',*,*,#54385,.F.);
#76441=ORIENTED_EDGE('',*,*,#54406,.T.);
#76442=ORIENTED_EDGE('',*,*,#54387,.F.);
#76443=ORIENTED_EDGE('',*,*,#54407,.T.);
#76444=ORIENTED_EDGE('',*,*,#54408,.T.);
#76445=ORIENTED_EDGE('',*,*,#54409,.T.);
#76446=ORIENTED_EDGE('',*,*,#54410,.F.);
#76447=ORIENTED_EDGE('',*,*,#54411,.F.);
#76448=ORIENTED_EDGE('',*,*,#54412,.F.);
#76449=ORIENTED_EDGE('',*,*,#54413,.T.);
#76450=ORIENTED_EDGE('',*,*,#54411,.T.);
#76451=ORIENTED_EDGE('',*,*,#54414,.T.);
#76452=ORIENTED_EDGE('',*,*,#54415,.T.);
#76453=ORIENTED_EDGE('',*,*,#54416,.T.);
#76454=ORIENTED_EDGE('',*,*,#54417,.T.);
#76455=ORIENTED_EDGE('',*,*,#54418,.T.);
#76456=ORIENTED_EDGE('',*,*,#54419,.T.);
#76457=ORIENTED_EDGE('',*,*,#54420,.T.);
#76458=ORIENTED_EDGE('',*,*,#54421,.T.);
#76459=ORIENTED_EDGE('',*,*,#54422,.T.);
#76460=ORIENTED_EDGE('',*,*,#54423,.F.);
#76461=ORIENTED_EDGE('',*,*,#54424,.F.);
#76462=ORIENTED_EDGE('',*,*,#54425,.F.);
#76463=ORIENTED_EDGE('',*,*,#54426,.T.);
#76464=ORIENTED_EDGE('',*,*,#54424,.T.);
#76465=ORIENTED_EDGE('',*,*,#54427,.T.);
#76466=ORIENTED_EDGE('',*,*,#54428,.T.);
#76467=ORIENTED_EDGE('',*,*,#54429,.T.);
#76468=ORIENTED_EDGE('',*,*,#52569,.F.);
#76469=ORIENTED_EDGE('',*,*,#54430,.T.);
#76470=ORIENTED_EDGE('',*,*,#54408,.F.);
#76471=ORIENTED_EDGE('',*,*,#54431,.T.);
#76472=ORIENTED_EDGE('',*,*,#54428,.F.);
#76473=ORIENTED_EDGE('',*,*,#54432,.T.);
#76474=ORIENTED_EDGE('',*,*,#52097,.F.);
#76475=ORIENTED_EDGE('',*,*,#54433,.T.);
#76476=ORIENTED_EDGE('',*,*,#54419,.F.);
#76477=ORIENTED_EDGE('',*,*,#54434,.T.);
#76478=ORIENTED_EDGE('',*,*,#54421,.F.);
#76479=ORIENTED_EDGE('',*,*,#54435,.T.);
#76480=ORIENTED_EDGE('',*,*,#54415,.F.);
#76481=ORIENTED_EDGE('',*,*,#54436,.T.);
#76482=ORIENTED_EDGE('',*,*,#54417,.F.);
#76483=ORIENTED_EDGE('',*,*,#54437,.T.);
#76484=ORIENTED_EDGE('',*,*,#54438,.T.);
#76485=ORIENTED_EDGE('',*,*,#54439,.T.);
#76486=ORIENTED_EDGE('',*,*,#54440,.F.);
#76487=ORIENTED_EDGE('',*,*,#54441,.F.);
#76488=ORIENTED_EDGE('',*,*,#54442,.F.);
#76489=ORIENTED_EDGE('',*,*,#54443,.T.);
#76490=ORIENTED_EDGE('',*,*,#54441,.T.);
#76491=ORIENTED_EDGE('',*,*,#54444,.T.);
#76492=ORIENTED_EDGE('',*,*,#54445,.T.);
#76493=ORIENTED_EDGE('',*,*,#54446,.T.);
#76494=ORIENTED_EDGE('',*,*,#54447,.T.);
#76495=ORIENTED_EDGE('',*,*,#54448,.T.);
#76496=ORIENTED_EDGE('',*,*,#54449,.T.);
#76497=ORIENTED_EDGE('',*,*,#54450,.T.);
#76498=ORIENTED_EDGE('',*,*,#54451,.T.);
#76499=ORIENTED_EDGE('',*,*,#54452,.T.);
#76500=ORIENTED_EDGE('',*,*,#54453,.F.);
#76501=ORIENTED_EDGE('',*,*,#54454,.F.);
#76502=ORIENTED_EDGE('',*,*,#54455,.F.);
#76503=ORIENTED_EDGE('',*,*,#54456,.T.);
#76504=ORIENTED_EDGE('',*,*,#54454,.T.);
#76505=ORIENTED_EDGE('',*,*,#54457,.T.);
#76506=ORIENTED_EDGE('',*,*,#54458,.T.);
#76507=ORIENTED_EDGE('',*,*,#54459,.T.);
#76508=ORIENTED_EDGE('',*,*,#52575,.F.);
#76509=ORIENTED_EDGE('',*,*,#54460,.T.);
#76510=ORIENTED_EDGE('',*,*,#54438,.F.);
#76511=ORIENTED_EDGE('',*,*,#54461,.T.);
#76512=ORIENTED_EDGE('',*,*,#54458,.F.);
#76513=ORIENTED_EDGE('',*,*,#54462,.T.);
#76514=ORIENTED_EDGE('',*,*,#52091,.F.);
#76515=ORIENTED_EDGE('',*,*,#54463,.T.);
#76516=ORIENTED_EDGE('',*,*,#54449,.F.);
#76517=ORIENTED_EDGE('',*,*,#54464,.T.);
#76518=ORIENTED_EDGE('',*,*,#54451,.F.);
#76519=ORIENTED_EDGE('',*,*,#54465,.T.);
#76520=ORIENTED_EDGE('',*,*,#54445,.F.);
#76521=ORIENTED_EDGE('',*,*,#54466,.T.);
#76522=ORIENTED_EDGE('',*,*,#54447,.F.);
#76523=ORIENTED_EDGE('',*,*,#54467,.T.);
#76524=ORIENTED_EDGE('',*,*,#54468,.T.);
#76525=ORIENTED_EDGE('',*,*,#54469,.T.);
#76526=ORIENTED_EDGE('',*,*,#54470,.F.);
#76527=ORIENTED_EDGE('',*,*,#54471,.F.);
#76528=ORIENTED_EDGE('',*,*,#54472,.F.);
#76529=ORIENTED_EDGE('',*,*,#54473,.T.);
#76530=ORIENTED_EDGE('',*,*,#54471,.T.);
#76531=ORIENTED_EDGE('',*,*,#54474,.T.);
#76532=ORIENTED_EDGE('',*,*,#54475,.T.);
#76533=ORIENTED_EDGE('',*,*,#54476,.T.);
#76534=ORIENTED_EDGE('',*,*,#54477,.T.);
#76535=ORIENTED_EDGE('',*,*,#54478,.T.);
#76536=ORIENTED_EDGE('',*,*,#54479,.T.);
#76537=ORIENTED_EDGE('',*,*,#54480,.T.);
#76538=ORIENTED_EDGE('',*,*,#54481,.T.);
#76539=ORIENTED_EDGE('',*,*,#54482,.T.);
#76540=ORIENTED_EDGE('',*,*,#54483,.F.);
#76541=ORIENTED_EDGE('',*,*,#54484,.F.);
#76542=ORIENTED_EDGE('',*,*,#54485,.F.);
#76543=ORIENTED_EDGE('',*,*,#54486,.T.);
#76544=ORIENTED_EDGE('',*,*,#54484,.T.);
#76545=ORIENTED_EDGE('',*,*,#54487,.T.);
#76546=ORIENTED_EDGE('',*,*,#54488,.T.);
#76547=ORIENTED_EDGE('',*,*,#54489,.T.);
#76548=ORIENTED_EDGE('',*,*,#52581,.F.);
#76549=ORIENTED_EDGE('',*,*,#54490,.T.);
#76550=ORIENTED_EDGE('',*,*,#54468,.F.);
#76551=ORIENTED_EDGE('',*,*,#54491,.T.);
#76552=ORIENTED_EDGE('',*,*,#54488,.F.);
#76553=ORIENTED_EDGE('',*,*,#54492,.T.);
#76554=ORIENTED_EDGE('',*,*,#52085,.F.);
#76555=ORIENTED_EDGE('',*,*,#54493,.T.);
#76556=ORIENTED_EDGE('',*,*,#54479,.F.);
#76557=ORIENTED_EDGE('',*,*,#54494,.T.);
#76558=ORIENTED_EDGE('',*,*,#54481,.F.);
#76559=ORIENTED_EDGE('',*,*,#54495,.T.);
#76560=ORIENTED_EDGE('',*,*,#54475,.F.);
#76561=ORIENTED_EDGE('',*,*,#54496,.T.);
#76562=ORIENTED_EDGE('',*,*,#54477,.F.);
#76563=ORIENTED_EDGE('',*,*,#54497,.T.);
#76564=ORIENTED_EDGE('',*,*,#54498,.T.);
#76565=ORIENTED_EDGE('',*,*,#54499,.T.);
#76566=ORIENTED_EDGE('',*,*,#54500,.F.);
#76567=ORIENTED_EDGE('',*,*,#54501,.F.);
#76568=ORIENTED_EDGE('',*,*,#54502,.F.);
#76569=ORIENTED_EDGE('',*,*,#54503,.T.);
#76570=ORIENTED_EDGE('',*,*,#54501,.T.);
#76571=ORIENTED_EDGE('',*,*,#54504,.T.);
#76572=ORIENTED_EDGE('',*,*,#54505,.T.);
#76573=ORIENTED_EDGE('',*,*,#54506,.T.);
#76574=ORIENTED_EDGE('',*,*,#54507,.T.);
#76575=ORIENTED_EDGE('',*,*,#54508,.T.);
#76576=ORIENTED_EDGE('',*,*,#54509,.T.);
#76577=ORIENTED_EDGE('',*,*,#54510,.T.);
#76578=ORIENTED_EDGE('',*,*,#54511,.T.);
#76579=ORIENTED_EDGE('',*,*,#54512,.T.);
#76580=ORIENTED_EDGE('',*,*,#54513,.F.);
#76581=ORIENTED_EDGE('',*,*,#54514,.F.);
#76582=ORIENTED_EDGE('',*,*,#54515,.F.);
#76583=ORIENTED_EDGE('',*,*,#54516,.T.);
#76584=ORIENTED_EDGE('',*,*,#54514,.T.);
#76585=ORIENTED_EDGE('',*,*,#54517,.T.);
#76586=ORIENTED_EDGE('',*,*,#54518,.T.);
#76587=ORIENTED_EDGE('',*,*,#54519,.T.);
#76588=ORIENTED_EDGE('',*,*,#52587,.F.);
#76589=ORIENTED_EDGE('',*,*,#54520,.T.);
#76590=ORIENTED_EDGE('',*,*,#54498,.F.);
#76591=ORIENTED_EDGE('',*,*,#54521,.T.);
#76592=ORIENTED_EDGE('',*,*,#54518,.F.);
#76593=ORIENTED_EDGE('',*,*,#54522,.T.);
#76594=ORIENTED_EDGE('',*,*,#52079,.F.);
#76595=ORIENTED_EDGE('',*,*,#54523,.T.);
#76596=ORIENTED_EDGE('',*,*,#54509,.F.);
#76597=ORIENTED_EDGE('',*,*,#54524,.T.);
#76598=ORIENTED_EDGE('',*,*,#54511,.F.);
#76599=ORIENTED_EDGE('',*,*,#54525,.T.);
#76600=ORIENTED_EDGE('',*,*,#54505,.F.);
#76601=ORIENTED_EDGE('',*,*,#54526,.T.);
#76602=ORIENTED_EDGE('',*,*,#54507,.F.);
#76603=ORIENTED_EDGE('',*,*,#54527,.T.);
#76604=ORIENTED_EDGE('',*,*,#54528,.T.);
#76605=ORIENTED_EDGE('',*,*,#54529,.T.);
#76606=ORIENTED_EDGE('',*,*,#54530,.F.);
#76607=ORIENTED_EDGE('',*,*,#54531,.F.);
#76608=ORIENTED_EDGE('',*,*,#54532,.F.);
#76609=ORIENTED_EDGE('',*,*,#54533,.T.);
#76610=ORIENTED_EDGE('',*,*,#54531,.T.);
#76611=ORIENTED_EDGE('',*,*,#54534,.T.);
#76612=ORIENTED_EDGE('',*,*,#54535,.T.);
#76613=ORIENTED_EDGE('',*,*,#54536,.T.);
#76614=ORIENTED_EDGE('',*,*,#54537,.T.);
#76615=ORIENTED_EDGE('',*,*,#54538,.T.);
#76616=ORIENTED_EDGE('',*,*,#54539,.T.);
#76617=ORIENTED_EDGE('',*,*,#54540,.T.);
#76618=ORIENTED_EDGE('',*,*,#54541,.T.);
#76619=ORIENTED_EDGE('',*,*,#54542,.T.);
#76620=ORIENTED_EDGE('',*,*,#54543,.F.);
#76621=ORIENTED_EDGE('',*,*,#54544,.F.);
#76622=ORIENTED_EDGE('',*,*,#54545,.F.);
#76623=ORIENTED_EDGE('',*,*,#54546,.T.);
#76624=ORIENTED_EDGE('',*,*,#54544,.T.);
#76625=ORIENTED_EDGE('',*,*,#54547,.T.);
#76626=ORIENTED_EDGE('',*,*,#54548,.T.);
#76627=ORIENTED_EDGE('',*,*,#54549,.T.);
#76628=ORIENTED_EDGE('',*,*,#52593,.F.);
#76629=ORIENTED_EDGE('',*,*,#54550,.T.);
#76630=ORIENTED_EDGE('',*,*,#54528,.F.);
#76631=ORIENTED_EDGE('',*,*,#54551,.T.);
#76632=ORIENTED_EDGE('',*,*,#54548,.F.);
#76633=ORIENTED_EDGE('',*,*,#54552,.T.);
#76634=ORIENTED_EDGE('',*,*,#52073,.F.);
#76635=ORIENTED_EDGE('',*,*,#54553,.T.);
#76636=ORIENTED_EDGE('',*,*,#54539,.F.);
#76637=ORIENTED_EDGE('',*,*,#54554,.T.);
#76638=ORIENTED_EDGE('',*,*,#54541,.F.);
#76639=ORIENTED_EDGE('',*,*,#54555,.T.);
#76640=ORIENTED_EDGE('',*,*,#54535,.F.);
#76641=ORIENTED_EDGE('',*,*,#54556,.T.);
#76642=ORIENTED_EDGE('',*,*,#54537,.F.);
#76643=ORIENTED_EDGE('',*,*,#54557,.T.);
#76644=ORIENTED_EDGE('',*,*,#52052,.T.);
#76645=ORIENTED_EDGE('',*,*,#52046,.T.);
#76646=ORIENTED_EDGE('',*,*,#54558,.T.);
#76647=ORIENTED_EDGE('',*,*,#54559,.T.);
#76648=ORIENTED_EDGE('',*,*,#54560,.F.);
#76649=ORIENTED_EDGE('',*,*,#54561,.F.);
#76650=ORIENTED_EDGE('',*,*,#54562,.F.);
#76651=ORIENTED_EDGE('',*,*,#54563,.T.);
#76652=ORIENTED_EDGE('',*,*,#54561,.T.);
#76653=ORIENTED_EDGE('',*,*,#54564,.T.);
#76654=ORIENTED_EDGE('',*,*,#54565,.T.);
#76655=ORIENTED_EDGE('',*,*,#54566,.T.);
#76656=ORIENTED_EDGE('',*,*,#54567,.T.);
#76657=ORIENTED_EDGE('',*,*,#54568,.T.);
#76658=ORIENTED_EDGE('',*,*,#54569,.T.);
#76659=ORIENTED_EDGE('',*,*,#54570,.T.);
#76660=ORIENTED_EDGE('',*,*,#54571,.T.);
#76661=ORIENTED_EDGE('',*,*,#54572,.T.);
#76662=ORIENTED_EDGE('',*,*,#54573,.F.);
#76663=ORIENTED_EDGE('',*,*,#54574,.F.);
#76664=ORIENTED_EDGE('',*,*,#54575,.F.);
#76665=ORIENTED_EDGE('',*,*,#54576,.T.);
#76666=ORIENTED_EDGE('',*,*,#54574,.T.);
#76667=ORIENTED_EDGE('',*,*,#54577,.T.);
#76668=ORIENTED_EDGE('',*,*,#54578,.T.);
#76669=ORIENTED_EDGE('',*,*,#54579,.T.);
#76670=ORIENTED_EDGE('',*,*,#52059,.T.);
#76671=ORIENTED_EDGE('',*,*,#52053,.T.);
#76672=ORIENTED_EDGE('',*,*,#52060,.T.);
#76673=ORIENTED_EDGE('',*,*,#52787,.F.);
#76674=ORIENTED_EDGE('',*,*,#52599,.F.);
#76675=ORIENTED_EDGE('',*,*,#54580,.T.);
#76676=ORIENTED_EDGE('',*,*,#54558,.F.);
#76677=ORIENTED_EDGE('',*,*,#54581,.T.);
#76678=ORIENTED_EDGE('',*,*,#54578,.F.);
#76679=ORIENTED_EDGE('',*,*,#54582,.T.);
#76680=ORIENTED_EDGE('',*,*,#52067,.F.);
#76681=ORIENTED_EDGE('',*,*,#54583,.T.);
#76682=ORIENTED_EDGE('',*,*,#54569,.F.);
#76683=ORIENTED_EDGE('',*,*,#54584,.T.);
#76684=ORIENTED_EDGE('',*,*,#54571,.F.);
#76685=ORIENTED_EDGE('',*,*,#54585,.T.);
#76686=ORIENTED_EDGE('',*,*,#54565,.F.);
#76687=ORIENTED_EDGE('',*,*,#54586,.T.);
#76688=ORIENTED_EDGE('',*,*,#54567,.F.);
#76689=ORIENTED_EDGE('',*,*,#54587,.T.);
#76690=ORIENTED_EDGE('',*,*,#54588,.T.);
#76691=ORIENTED_EDGE('',*,*,#54589,.T.);
#76692=ORIENTED_EDGE('',*,*,#54590,.T.);
#76693=ORIENTED_EDGE('',*,*,#54591,.T.);
#76694=ORIENTED_EDGE('',*,*,#54592,.T.);
#76695=ORIENTED_EDGE('',*,*,#54593,.T.);
#76696=ORIENTED_EDGE('',*,*,#54594,.T.);
#76697=ORIENTED_EDGE('',*,*,#54595,.T.);
#76698=ORIENTED_EDGE('',*,*,#54596,.T.);
#76699=ORIENTED_EDGE('',*,*,#54597,.T.);
#76700=ORIENTED_EDGE('',*,*,#54598,.T.);
#76701=ORIENTED_EDGE('',*,*,#54599,.T.);
#76702=ORIENTED_EDGE('',*,*,#54600,.T.);
#76703=ORIENTED_EDGE('',*,*,#54601,.T.);
#76704=ORIENTED_EDGE('',*,*,#54602,.T.);
#76705=ORIENTED_EDGE('',*,*,#54603,.T.);
#76706=ORIENTED_EDGE('',*,*,#54604,.T.);
#76707=ORIENTED_EDGE('',*,*,#54605,.T.);
#76708=ORIENTED_EDGE('',*,*,#54606,.T.);
#76709=ORIENTED_EDGE('',*,*,#54607,.T.);
#76710=ORIENTED_EDGE('',*,*,#54608,.T.);
#76711=ORIENTED_EDGE('',*,*,#54609,.T.);
#76712=ORIENTED_EDGE('',*,*,#54610,.T.);
#76713=ORIENTED_EDGE('',*,*,#54611,.T.);
#76714=ORIENTED_EDGE('',*,*,#54612,.T.);
#76715=ORIENTED_EDGE('',*,*,#54613,.T.);
#76716=ORIENTED_EDGE('',*,*,#54614,.T.);
#76717=ORIENTED_EDGE('',*,*,#54615,.T.);
#76718=ORIENTED_EDGE('',*,*,#54606,.F.);
#76719=ORIENTED_EDGE('',*,*,#54616,.T.);
#76720=ORIENTED_EDGE('',*,*,#54588,.F.);
#76721=ORIENTED_EDGE('',*,*,#54617,.T.);
#76722=ORIENTED_EDGE('',*,*,#54590,.F.);
#76723=ORIENTED_EDGE('',*,*,#54618,.T.);
#76724=ORIENTED_EDGE('',*,*,#54594,.F.);
#76725=ORIENTED_EDGE('',*,*,#54619,.T.);
#76726=ORIENTED_EDGE('',*,*,#54620,.F.);
#76727=ORIENTED_EDGE('',*,*,#54614,.F.);
#76728=ORIENTED_EDGE('',*,*,#54621,.F.);
#76729=ORIENTED_EDGE('',*,*,#54576,.F.);
#76730=ORIENTED_EDGE('',*,*,#54621,.T.);
#76731=ORIENTED_EDGE('',*,*,#54613,.F.);
#76732=ORIENTED_EDGE('',*,*,#54622,.F.);
#76733=ORIENTED_EDGE('',*,*,#54585,.F.);
#76734=ORIENTED_EDGE('',*,*,#54575,.T.);
#76735=ORIENTED_EDGE('',*,*,#54579,.F.);
#76736=ORIENTED_EDGE('',*,*,#54623,.F.);
#76737=ORIENTED_EDGE('',*,*,#54615,.F.);
#76738=ORIENTED_EDGE('',*,*,#54620,.T.);
#76739=ORIENTED_EDGE('',*,*,#54622,.T.);
#76740=ORIENTED_EDGE('',*,*,#54612,.F.);
#76741=ORIENTED_EDGE('',*,*,#54624,.F.);
#76742=ORIENTED_EDGE('',*,*,#54570,.F.);
#76743=ORIENTED_EDGE('',*,*,#54623,.T.);
#76744=ORIENTED_EDGE('',*,*,#54583,.F.);
#76745=ORIENTED_EDGE('',*,*,#54625,.F.);
#76746=ORIENTED_EDGE('',*,*,#54604,.F.);
#76747=ORIENTED_EDGE('',*,*,#54624,.T.);
#76748=ORIENTED_EDGE('',*,*,#54611,.F.);
#76749=ORIENTED_EDGE('',*,*,#54626,.F.);
#76750=ORIENTED_EDGE('',*,*,#54587,.F.);
#76751=ORIENTED_EDGE('',*,*,#54625,.T.);
#76752=ORIENTED_EDGE('',*,*,#52066,.F.);
#76753=ORIENTED_EDGE('',*,*,#54627,.F.);
#76754=ORIENTED_EDGE('',*,*,#54605,.F.);
#76755=ORIENTED_EDGE('',*,*,#54626,.T.);
#76756=ORIENTED_EDGE('',*,*,#54610,.F.);
#76757=ORIENTED_EDGE('',*,*,#54628,.F.);
#76758=ORIENTED_EDGE('',*,*,#54562,.T.);
#76759=ORIENTED_EDGE('',*,*,#54566,.F.);
#76760=ORIENTED_EDGE('',*,*,#54627,.T.);
#76761=ORIENTED_EDGE('',*,*,#52065,.F.);
#76762=ORIENTED_EDGE('',*,*,#54629,.F.);
#76763=ORIENTED_EDGE('',*,*,#54616,.F.);
#76764=ORIENTED_EDGE('',*,*,#54628,.T.);
#76765=ORIENTED_EDGE('',*,*,#54609,.F.);
#76766=ORIENTED_EDGE('',*,*,#54630,.F.);
#76767=ORIENTED_EDGE('',*,*,#54563,.F.);
#76768=ORIENTED_EDGE('',*,*,#54629,.T.);
#76769=ORIENTED_EDGE('',*,*,#52064,.F.);
#76770=ORIENTED_EDGE('',*,*,#54631,.F.);
#76771=ORIENTED_EDGE('',*,*,#54589,.F.);
#76772=ORIENTED_EDGE('',*,*,#54630,.T.);
#76773=ORIENTED_EDGE('',*,*,#54608,.F.);
#76774=ORIENTED_EDGE('',*,*,#54632,.F.);
#76775=ORIENTED_EDGE('',*,*,#54581,.F.);
#76776=ORIENTED_EDGE('',*,*,#54631,.T.);
#76777=ORIENTED_EDGE('',*,*,#52422,.F.);
#76778=ORIENTED_EDGE('',*,*,#54633,.F.);
#76779=ORIENTED_EDGE('',*,*,#54618,.F.);
#76780=ORIENTED_EDGE('',*,*,#54632,.T.);
#76781=ORIENTED_EDGE('',*,*,#54607,.F.);
#76782=ORIENTED_EDGE('',*,*,#54634,.F.);
#76783=ORIENTED_EDGE('',*,*,#52600,.F.);
#76784=ORIENTED_EDGE('',*,*,#54633,.T.);
#76785=ORIENTED_EDGE('',*,*,#52421,.F.);
#76786=ORIENTED_EDGE('',*,*,#54635,.F.);
#76787=ORIENTED_EDGE('',*,*,#54595,.F.);
#76788=ORIENTED_EDGE('',*,*,#54634,.T.);
#76789=ORIENTED_EDGE('',*,*,#54617,.F.);
#76790=ORIENTED_EDGE('',*,*,#54636,.F.);
#76791=ORIENTED_EDGE('',*,*,#52601,.F.);
#76792=ORIENTED_EDGE('',*,*,#54635,.T.);
#76793=ORIENTED_EDGE('',*,*,#52813,.F.);
#76794=ORIENTED_EDGE('',*,*,#54637,.F.);
#76795=ORIENTED_EDGE('',*,*,#54596,.F.);
#76796=ORIENTED_EDGE('',*,*,#54636,.T.);
#76797=ORIENTED_EDGE('',*,*,#54591,.F.);
#76798=ORIENTED_EDGE('',*,*,#54638,.F.);
#76799=ORIENTED_EDGE('',*,*,#52604,.F.);
#76800=ORIENTED_EDGE('',*,*,#52602,.F.);
#76801=ORIENTED_EDGE('',*,*,#52809,.F.);
#76802=ORIENTED_EDGE('',*,*,#52805,.T.);
#76803=ORIENTED_EDGE('',*,*,#54639,.F.);
#76804=ORIENTED_EDGE('',*,*,#54597,.F.);
#76805=ORIENTED_EDGE('',*,*,#54637,.T.);
#76806=ORIENTED_EDGE('',*,*,#54638,.T.);
#76807=ORIENTED_EDGE('',*,*,#54619,.F.);
#76808=ORIENTED_EDGE('',*,*,#54640,.F.);
#76809=ORIENTED_EDGE('',*,*,#52605,.F.);
#76810=ORIENTED_EDGE('',*,*,#54639,.T.);
#76811=ORIENTED_EDGE('',*,*,#52804,.F.);
#76812=ORIENTED_EDGE('',*,*,#54641,.F.);
#76813=ORIENTED_EDGE('',*,*,#54598,.F.);
#76814=ORIENTED_EDGE('',*,*,#54640,.T.);
#76815=ORIENTED_EDGE('',*,*,#54593,.F.);
#76816=ORIENTED_EDGE('',*,*,#54642,.F.);
#76817=ORIENTED_EDGE('',*,*,#52606,.F.);
#76818=ORIENTED_EDGE('',*,*,#54641,.T.);
#76819=ORIENTED_EDGE('',*,*,#52815,.F.);
#76820=ORIENTED_EDGE('',*,*,#54643,.F.);
#76821=ORIENTED_EDGE('',*,*,#54599,.F.);
#76822=ORIENTED_EDGE('',*,*,#54642,.T.);
#76823=ORIENTED_EDGE('',*,*,#54592,.F.);
#76824=ORIENTED_EDGE('',*,*,#54644,.F.);
#76825=ORIENTED_EDGE('',*,*,#52811,.F.);
#76826=ORIENTED_EDGE('',*,*,#54643,.T.);
#76827=ORIENTED_EDGE('',*,*,#52800,.F.);
#76828=ORIENTED_EDGE('',*,*,#54645,.F.);
#76829=ORIENTED_EDGE('',*,*,#54600,.F.);
#76830=ORIENTED_EDGE('',*,*,#54644,.T.);
#76831=ORIENTED_EDGE('',*,*,#54603,.F.);
#76832=ORIENTED_EDGE('',*,*,#54646,.F.);
#76833=ORIENTED_EDGE('',*,*,#52791,.F.);
#76834=ORIENTED_EDGE('',*,*,#54645,.T.);
#76835=ORIENTED_EDGE('',*,*,#52817,.F.);
#76836=ORIENTED_EDGE('',*,*,#54647,.F.);
#76837=ORIENTED_EDGE('',*,*,#54601,.F.);
#76838=ORIENTED_EDGE('',*,*,#54646,.T.);
#76839=ORIENTED_EDGE('',*,*,#54602,.F.);
#76840=ORIENTED_EDGE('',*,*,#54647,.T.);
#76841=ORIENTED_EDGE('',*,*,#52796,.F.);
#76842=ORIENTED_EDGE('',*,*,#52792,.T.);
#76843=ORIENTED_EDGE('',*,*,#54648,.T.);
#76844=ORIENTED_EDGE('',*,*,#54649,.T.);
#76845=ORIENTED_EDGE('',*,*,#54650,.T.);
#76846=ORIENTED_EDGE('',*,*,#54651,.T.);
#76847=ORIENTED_EDGE('',*,*,#54652,.T.);
#76848=ORIENTED_EDGE('',*,*,#54653,.T.);
#76849=ORIENTED_EDGE('',*,*,#54654,.T.);
#76850=ORIENTED_EDGE('',*,*,#54655,.T.);
#76851=ORIENTED_EDGE('',*,*,#54656,.T.);
#76852=ORIENTED_EDGE('',*,*,#54657,.T.);
#76853=ORIENTED_EDGE('',*,*,#54658,.T.);
#76854=ORIENTED_EDGE('',*,*,#54659,.T.);
#76855=ORIENTED_EDGE('',*,*,#54660,.T.);
#76856=ORIENTED_EDGE('',*,*,#54661,.T.);
#76857=ORIENTED_EDGE('',*,*,#54662,.T.);
#76858=ORIENTED_EDGE('',*,*,#54663,.T.);
#76859=ORIENTED_EDGE('',*,*,#54664,.T.);
#76860=ORIENTED_EDGE('',*,*,#54665,.T.);
#76861=ORIENTED_EDGE('',*,*,#54666,.T.);
#76862=ORIENTED_EDGE('',*,*,#54667,.T.);
#76863=ORIENTED_EDGE('',*,*,#54668,.T.);
#76864=ORIENTED_EDGE('',*,*,#54669,.T.);
#76865=ORIENTED_EDGE('',*,*,#54670,.T.);
#76866=ORIENTED_EDGE('',*,*,#54671,.T.);
#76867=ORIENTED_EDGE('',*,*,#54672,.T.);
#76868=ORIENTED_EDGE('',*,*,#54673,.T.);
#76869=ORIENTED_EDGE('',*,*,#54674,.T.);
#76870=ORIENTED_EDGE('',*,*,#54675,.T.);
#76871=ORIENTED_EDGE('',*,*,#54676,.T.);
#76872=ORIENTED_EDGE('',*,*,#54677,.T.);
#76873=ORIENTED_EDGE('',*,*,#54678,.T.);
#76874=ORIENTED_EDGE('',*,*,#54679,.T.);
#76875=ORIENTED_EDGE('',*,*,#54680,.T.);
#76876=ORIENTED_EDGE('',*,*,#54681,.T.);
#76877=ORIENTED_EDGE('',*,*,#54682,.T.);
#76878=ORIENTED_EDGE('',*,*,#54683,.T.);
#76879=ORIENTED_EDGE('',*,*,#54684,.T.);
#76880=ORIENTED_EDGE('',*,*,#54685,.T.);
#76881=ORIENTED_EDGE('',*,*,#54686,.T.);
#76882=ORIENTED_EDGE('',*,*,#54687,.T.);
#76883=ORIENTED_EDGE('',*,*,#54688,.T.);
#76884=ORIENTED_EDGE('',*,*,#54689,.T.);
#76885=ORIENTED_EDGE('',*,*,#54690,.T.);
#76886=ORIENTED_EDGE('',*,*,#54691,.T.);
#76887=ORIENTED_EDGE('',*,*,#54692,.T.);
#76888=ORIENTED_EDGE('',*,*,#54693,.T.);
#76889=ORIENTED_EDGE('',*,*,#54694,.T.);
#76890=ORIENTED_EDGE('',*,*,#54695,.T.);
#76891=ORIENTED_EDGE('',*,*,#54696,.T.);
#76892=ORIENTED_EDGE('',*,*,#54697,.T.);
#76893=ORIENTED_EDGE('',*,*,#54698,.T.);
#76894=ORIENTED_EDGE('',*,*,#54699,.T.);
#76895=ORIENTED_EDGE('',*,*,#54700,.T.);
#76896=ORIENTED_EDGE('',*,*,#54701,.T.);
#76897=ORIENTED_EDGE('',*,*,#54702,.T.);
#76898=ORIENTED_EDGE('',*,*,#54703,.T.);
#76899=ORIENTED_EDGE('',*,*,#54704,.T.);
#76900=ORIENTED_EDGE('',*,*,#54705,.T.);
#76901=ORIENTED_EDGE('',*,*,#54706,.T.);
#76902=ORIENTED_EDGE('',*,*,#54707,.T.);
#76903=ORIENTED_EDGE('',*,*,#54708,.T.);
#76904=ORIENTED_EDGE('',*,*,#54709,.T.);
#76905=ORIENTED_EDGE('',*,*,#54710,.T.);
#76906=ORIENTED_EDGE('',*,*,#54711,.T.);
#76907=ORIENTED_EDGE('',*,*,#54712,.T.);
#76908=ORIENTED_EDGE('',*,*,#54713,.T.);
#76909=ORIENTED_EDGE('',*,*,#54714,.T.);
#76910=ORIENTED_EDGE('',*,*,#54715,.T.);
#76911=ORIENTED_EDGE('',*,*,#54716,.T.);
#76912=ORIENTED_EDGE('',*,*,#54717,.T.);
#76913=ORIENTED_EDGE('',*,*,#54718,.T.);
#76914=ORIENTED_EDGE('',*,*,#54719,.T.);
#76915=ORIENTED_EDGE('',*,*,#54720,.T.);
#76916=ORIENTED_EDGE('',*,*,#54721,.T.);
#76917=ORIENTED_EDGE('',*,*,#54722,.T.);
#76918=ORIENTED_EDGE('',*,*,#54723,.T.);
#76919=ORIENTED_EDGE('',*,*,#54724,.T.);
#76920=ORIENTED_EDGE('',*,*,#54725,.T.);
#76921=ORIENTED_EDGE('',*,*,#54726,.T.);
#76922=ORIENTED_EDGE('',*,*,#54727,.T.);
#76923=ORIENTED_EDGE('',*,*,#54728,.T.);
#76924=ORIENTED_EDGE('',*,*,#54729,.T.);
#76925=ORIENTED_EDGE('',*,*,#54730,.T.);
#76926=ORIENTED_EDGE('',*,*,#54731,.T.);
#76927=ORIENTED_EDGE('',*,*,#54732,.T.);
#76928=ORIENTED_EDGE('',*,*,#54733,.T.);
#76929=ORIENTED_EDGE('',*,*,#54734,.T.);
#76930=ORIENTED_EDGE('',*,*,#54735,.T.);
#76931=ORIENTED_EDGE('',*,*,#54736,.T.);
#76932=ORIENTED_EDGE('',*,*,#54737,.T.);
#76933=ORIENTED_EDGE('',*,*,#54738,.T.);
#76934=ORIENTED_EDGE('',*,*,#54739,.T.);
#76935=ORIENTED_EDGE('',*,*,#54740,.T.);
#76936=ORIENTED_EDGE('',*,*,#54741,.T.);
#76937=ORIENTED_EDGE('',*,*,#54742,.T.);
#76938=ORIENTED_EDGE('',*,*,#54743,.T.);
#76939=ORIENTED_EDGE('',*,*,#54744,.T.);
#76940=ORIENTED_EDGE('',*,*,#54745,.T.);
#76941=ORIENTED_EDGE('',*,*,#54746,.T.);
#76942=ORIENTED_EDGE('',*,*,#54747,.T.);
#76943=ORIENTED_EDGE('',*,*,#54748,.T.);
#76944=ORIENTED_EDGE('',*,*,#54749,.T.);
#76945=ORIENTED_EDGE('',*,*,#54750,.T.);
#76946=ORIENTED_EDGE('',*,*,#54751,.T.);
#76947=ORIENTED_EDGE('',*,*,#54752,.T.);
#76948=ORIENTED_EDGE('',*,*,#54753,.T.);
#76949=ORIENTED_EDGE('',*,*,#54754,.T.);
#76950=ORIENTED_EDGE('',*,*,#54755,.T.);
#76951=ORIENTED_EDGE('',*,*,#54756,.T.);
#76952=ORIENTED_EDGE('',*,*,#54757,.T.);
#76953=ORIENTED_EDGE('',*,*,#54758,.T.);
#76954=ORIENTED_EDGE('',*,*,#54759,.T.);
#76955=ORIENTED_EDGE('',*,*,#54760,.T.);
#76956=ORIENTED_EDGE('',*,*,#54761,.T.);
#76957=ORIENTED_EDGE('',*,*,#54762,.T.);
#76958=ORIENTED_EDGE('',*,*,#54763,.T.);
#76959=ORIENTED_EDGE('',*,*,#54764,.T.);
#76960=ORIENTED_EDGE('',*,*,#54765,.T.);
#76961=ORIENTED_EDGE('',*,*,#54766,.T.);
#76962=ORIENTED_EDGE('',*,*,#54767,.T.);
#76963=ORIENTED_EDGE('',*,*,#54768,.T.);
#76964=ORIENTED_EDGE('',*,*,#54769,.T.);
#76965=ORIENTED_EDGE('',*,*,#54770,.T.);
#76966=ORIENTED_EDGE('',*,*,#54771,.T.);
#76967=ORIENTED_EDGE('',*,*,#54772,.T.);
#76968=ORIENTED_EDGE('',*,*,#54773,.T.);
#76969=ORIENTED_EDGE('',*,*,#54774,.T.);
#76970=ORIENTED_EDGE('',*,*,#54775,.T.);
#76971=ORIENTED_EDGE('',*,*,#54776,.T.);
#76972=ORIENTED_EDGE('',*,*,#54777,.T.);
#76973=ORIENTED_EDGE('',*,*,#54778,.T.);
#76974=ORIENTED_EDGE('',*,*,#54779,.T.);
#76975=ORIENTED_EDGE('',*,*,#54780,.T.);
#76976=ORIENTED_EDGE('',*,*,#54781,.T.);
#76977=ORIENTED_EDGE('',*,*,#54782,.T.);
#76978=ORIENTED_EDGE('',*,*,#54783,.T.);
#76979=ORIENTED_EDGE('',*,*,#54784,.T.);
#76980=ORIENTED_EDGE('',*,*,#54785,.T.);
#76981=ORIENTED_EDGE('',*,*,#54786,.T.);
#76982=ORIENTED_EDGE('',*,*,#54787,.T.);
#76983=ORIENTED_EDGE('',*,*,#54788,.T.);
#76984=ORIENTED_EDGE('',*,*,#54789,.T.);
#76985=ORIENTED_EDGE('',*,*,#54790,.T.);
#76986=ORIENTED_EDGE('',*,*,#54791,.T.);
#76987=ORIENTED_EDGE('',*,*,#54792,.T.);
#76988=ORIENTED_EDGE('',*,*,#54793,.T.);
#76989=ORIENTED_EDGE('',*,*,#54794,.T.);
#76990=ORIENTED_EDGE('',*,*,#54795,.T.);
#76991=ORIENTED_EDGE('',*,*,#54796,.T.);
#76992=ORIENTED_EDGE('',*,*,#54797,.T.);
#76993=ORIENTED_EDGE('',*,*,#54798,.T.);
#76994=ORIENTED_EDGE('',*,*,#54799,.T.);
#76995=ORIENTED_EDGE('',*,*,#54800,.T.);
#76996=ORIENTED_EDGE('',*,*,#54801,.T.);
#76997=ORIENTED_EDGE('',*,*,#54802,.T.);
#76998=ORIENTED_EDGE('',*,*,#54803,.T.);
#76999=ORIENTED_EDGE('',*,*,#54804,.T.);
#77000=ORIENTED_EDGE('',*,*,#54805,.T.);
#77001=ORIENTED_EDGE('',*,*,#54806,.T.);
#77002=ORIENTED_EDGE('',*,*,#54807,.T.);
#77003=ORIENTED_EDGE('',*,*,#54808,.T.);
#77004=ORIENTED_EDGE('',*,*,#54809,.T.);
#77005=ORIENTED_EDGE('',*,*,#54810,.T.);
#77006=ORIENTED_EDGE('',*,*,#54811,.T.);
#77007=ORIENTED_EDGE('',*,*,#54812,.T.);
#77008=ORIENTED_EDGE('',*,*,#54813,.T.);
#77009=ORIENTED_EDGE('',*,*,#54814,.T.);
#77010=ORIENTED_EDGE('',*,*,#54815,.T.);
#77011=ORIENTED_EDGE('',*,*,#54816,.T.);
#77012=ORIENTED_EDGE('',*,*,#54817,.T.);
#77013=ORIENTED_EDGE('',*,*,#54818,.T.);
#77014=ORIENTED_EDGE('',*,*,#54819,.T.);
#77015=ORIENTED_EDGE('',*,*,#54820,.T.);
#77016=ORIENTED_EDGE('',*,*,#54821,.T.);
#77017=ORIENTED_EDGE('',*,*,#54822,.T.);
#77018=ORIENTED_EDGE('',*,*,#54823,.T.);
#77019=ORIENTED_EDGE('',*,*,#54824,.T.);
#77020=ORIENTED_EDGE('',*,*,#54825,.T.);
#77021=ORIENTED_EDGE('',*,*,#54826,.T.);
#77022=ORIENTED_EDGE('',*,*,#54827,.T.);
#77023=ORIENTED_EDGE('',*,*,#54828,.T.);
#77024=ORIENTED_EDGE('',*,*,#54829,.T.);
#77025=ORIENTED_EDGE('',*,*,#54830,.T.);
#77026=ORIENTED_EDGE('',*,*,#54831,.T.);
#77027=ORIENTED_EDGE('',*,*,#54832,.T.);
#77028=ORIENTED_EDGE('',*,*,#54833,.T.);
#77029=ORIENTED_EDGE('',*,*,#54834,.T.);
#77030=ORIENTED_EDGE('',*,*,#54835,.T.);
#77031=ORIENTED_EDGE('',*,*,#54836,.T.);
#77032=ORIENTED_EDGE('',*,*,#54837,.T.);
#77033=ORIENTED_EDGE('',*,*,#54838,.T.);
#77034=ORIENTED_EDGE('',*,*,#54839,.T.);
#77035=ORIENTED_EDGE('',*,*,#54840,.T.);
#77036=ORIENTED_EDGE('',*,*,#54841,.T.);
#77037=ORIENTED_EDGE('',*,*,#54842,.T.);
#77038=ORIENTED_EDGE('',*,*,#54843,.T.);
#77039=ORIENTED_EDGE('',*,*,#54844,.T.);
#77040=ORIENTED_EDGE('',*,*,#54845,.T.);
#77041=ORIENTED_EDGE('',*,*,#54846,.T.);
#77042=ORIENTED_EDGE('',*,*,#54847,.T.);
#77043=ORIENTED_EDGE('',*,*,#54848,.T.);
#77044=ORIENTED_EDGE('',*,*,#54849,.T.);
#77045=ORIENTED_EDGE('',*,*,#54850,.T.);
#77046=ORIENTED_EDGE('',*,*,#54851,.T.);
#77047=ORIENTED_EDGE('',*,*,#54852,.T.);
#77048=ORIENTED_EDGE('',*,*,#54853,.T.);
#77049=ORIENTED_EDGE('',*,*,#54854,.T.);
#77050=ORIENTED_EDGE('',*,*,#54855,.T.);
#77051=ORIENTED_EDGE('',*,*,#54856,.T.);
#77052=ORIENTED_EDGE('',*,*,#54857,.T.);
#77053=ORIENTED_EDGE('',*,*,#54858,.T.);
#77054=ORIENTED_EDGE('',*,*,#54859,.T.);
#77055=ORIENTED_EDGE('',*,*,#54860,.T.);
#77056=ORIENTED_EDGE('',*,*,#54861,.T.);
#77057=ORIENTED_EDGE('',*,*,#54862,.T.);
#77058=ORIENTED_EDGE('',*,*,#54863,.T.);
#77059=ORIENTED_EDGE('',*,*,#54864,.T.);
#77060=ORIENTED_EDGE('',*,*,#54865,.T.);
#77061=ORIENTED_EDGE('',*,*,#54866,.T.);
#77062=ORIENTED_EDGE('',*,*,#54867,.T.);
#77063=ORIENTED_EDGE('',*,*,#54868,.T.);
#77064=ORIENTED_EDGE('',*,*,#54869,.T.);
#77065=ORIENTED_EDGE('',*,*,#54870,.T.);
#77066=ORIENTED_EDGE('',*,*,#54871,.T.);
#77067=ORIENTED_EDGE('',*,*,#54872,.T.);
#77068=ORIENTED_EDGE('',*,*,#54873,.T.);
#77069=ORIENTED_EDGE('',*,*,#54874,.T.);
#77070=ORIENTED_EDGE('',*,*,#54875,.T.);
#77071=ORIENTED_EDGE('',*,*,#54876,.T.);
#77072=ORIENTED_EDGE('',*,*,#54877,.T.);
#77073=ORIENTED_EDGE('',*,*,#54878,.T.);
#77074=ORIENTED_EDGE('',*,*,#54879,.T.);
#77075=ORIENTED_EDGE('',*,*,#54880,.T.);
#77076=ORIENTED_EDGE('',*,*,#54881,.T.);
#77077=ORIENTED_EDGE('',*,*,#54882,.T.);
#77078=ORIENTED_EDGE('',*,*,#54883,.T.);
#77079=ORIENTED_EDGE('',*,*,#54884,.T.);
#77080=ORIENTED_EDGE('',*,*,#54885,.T.);
#77081=ORIENTED_EDGE('',*,*,#54886,.T.);
#77082=ORIENTED_EDGE('',*,*,#54887,.T.);
#77083=ORIENTED_EDGE('',*,*,#54888,.T.);
#77084=ORIENTED_EDGE('',*,*,#54889,.T.);
#77085=ORIENTED_EDGE('',*,*,#54890,.T.);
#77086=ORIENTED_EDGE('',*,*,#54891,.T.);
#77087=ORIENTED_EDGE('',*,*,#54892,.T.);
#77088=ORIENTED_EDGE('',*,*,#54893,.T.);
#77089=ORIENTED_EDGE('',*,*,#54894,.T.);
#77090=ORIENTED_EDGE('',*,*,#54895,.T.);
#77091=ORIENTED_EDGE('',*,*,#54896,.T.);
#77092=ORIENTED_EDGE('',*,*,#54897,.T.);
#77093=ORIENTED_EDGE('',*,*,#54898,.T.);
#77094=ORIENTED_EDGE('',*,*,#54899,.T.);
#77095=ORIENTED_EDGE('',*,*,#54900,.T.);
#77096=ORIENTED_EDGE('',*,*,#54901,.T.);
#77097=ORIENTED_EDGE('',*,*,#54902,.T.);
#77098=ORIENTED_EDGE('',*,*,#54903,.T.);
#77099=ORIENTED_EDGE('',*,*,#54904,.T.);
#77100=ORIENTED_EDGE('',*,*,#54905,.T.);
#77101=ORIENTED_EDGE('',*,*,#54906,.T.);
#77102=ORIENTED_EDGE('',*,*,#54907,.T.);
#77103=ORIENTED_EDGE('',*,*,#54908,.T.);
#77104=ORIENTED_EDGE('',*,*,#54909,.T.);
#77105=ORIENTED_EDGE('',*,*,#54910,.T.);
#77106=ORIENTED_EDGE('',*,*,#54911,.T.);
#77107=ORIENTED_EDGE('',*,*,#54912,.T.);
#77108=ORIENTED_EDGE('',*,*,#54913,.T.);
#77109=ORIENTED_EDGE('',*,*,#54914,.T.);
#77110=ORIENTED_EDGE('',*,*,#54915,.T.);
#77111=ORIENTED_EDGE('',*,*,#54916,.T.);
#77112=ORIENTED_EDGE('',*,*,#54917,.T.);
#77113=ORIENTED_EDGE('',*,*,#54918,.T.);
#77114=ORIENTED_EDGE('',*,*,#54919,.T.);
#77115=ORIENTED_EDGE('',*,*,#54920,.T.);
#77116=ORIENTED_EDGE('',*,*,#54921,.T.);
#77117=ORIENTED_EDGE('',*,*,#54922,.T.);
#77118=ORIENTED_EDGE('',*,*,#54923,.T.);
#77119=ORIENTED_EDGE('',*,*,#54924,.T.);
#77120=ORIENTED_EDGE('',*,*,#54925,.T.);
#77121=ORIENTED_EDGE('',*,*,#54926,.T.);
#77122=ORIENTED_EDGE('',*,*,#54927,.T.);
#77123=ORIENTED_EDGE('',*,*,#54928,.T.);
#77124=ORIENTED_EDGE('',*,*,#54929,.T.);
#77125=ORIENTED_EDGE('',*,*,#54930,.T.);
#77126=ORIENTED_EDGE('',*,*,#54931,.T.);
#77127=ORIENTED_EDGE('',*,*,#54932,.T.);
#77128=ORIENTED_EDGE('',*,*,#54933,.T.);
#77129=ORIENTED_EDGE('',*,*,#54934,.T.);
#77130=ORIENTED_EDGE('',*,*,#54935,.T.);
#77131=ORIENTED_EDGE('',*,*,#54936,.T.);
#77132=ORIENTED_EDGE('',*,*,#54937,.T.);
#77133=ORIENTED_EDGE('',*,*,#54938,.T.);
#77134=ORIENTED_EDGE('',*,*,#54939,.T.);
#77135=ORIENTED_EDGE('',*,*,#54940,.T.);
#77136=ORIENTED_EDGE('',*,*,#54941,.T.);
#77137=ORIENTED_EDGE('',*,*,#54942,.T.);
#77138=ORIENTED_EDGE('',*,*,#54943,.T.);
#77139=ORIENTED_EDGE('',*,*,#54944,.T.);
#77140=ORIENTED_EDGE('',*,*,#54945,.T.);
#77141=ORIENTED_EDGE('',*,*,#54946,.T.);
#77142=ORIENTED_EDGE('',*,*,#54947,.T.);
#77143=ORIENTED_EDGE('',*,*,#54948,.T.);
#77144=ORIENTED_EDGE('',*,*,#54949,.T.);
#77145=ORIENTED_EDGE('',*,*,#54950,.T.);
#77146=ORIENTED_EDGE('',*,*,#54951,.T.);
#77147=ORIENTED_EDGE('',*,*,#54952,.T.);
#77148=ORIENTED_EDGE('',*,*,#54953,.T.);
#77149=ORIENTED_EDGE('',*,*,#54954,.T.);
#77150=ORIENTED_EDGE('',*,*,#54955,.T.);
#77151=ORIENTED_EDGE('',*,*,#54956,.T.);
#77152=ORIENTED_EDGE('',*,*,#54957,.T.);
#77153=ORIENTED_EDGE('',*,*,#54958,.T.);
#77154=ORIENTED_EDGE('',*,*,#54959,.T.);
#77155=ORIENTED_EDGE('',*,*,#54960,.T.);
#77156=ORIENTED_EDGE('',*,*,#54961,.T.);
#77157=ORIENTED_EDGE('',*,*,#54962,.T.);
#77158=ORIENTED_EDGE('',*,*,#54963,.T.);
#77159=ORIENTED_EDGE('',*,*,#54964,.T.);
#77160=ORIENTED_EDGE('',*,*,#54965,.T.);
#77161=ORIENTED_EDGE('',*,*,#54966,.T.);
#77162=ORIENTED_EDGE('',*,*,#54967,.T.);
#77163=ORIENTED_EDGE('',*,*,#54968,.T.);
#77164=ORIENTED_EDGE('',*,*,#54969,.T.);
#77165=ORIENTED_EDGE('',*,*,#54970,.T.);
#77166=ORIENTED_EDGE('',*,*,#54971,.T.);
#77167=ORIENTED_EDGE('',*,*,#54972,.T.);
#77168=ORIENTED_EDGE('',*,*,#54973,.T.);
#77169=ORIENTED_EDGE('',*,*,#54974,.T.);
#77170=ORIENTED_EDGE('',*,*,#54975,.T.);
#77171=ORIENTED_EDGE('',*,*,#54976,.T.);
#77172=ORIENTED_EDGE('',*,*,#54977,.T.);
#77173=ORIENTED_EDGE('',*,*,#54978,.T.);
#77174=ORIENTED_EDGE('',*,*,#54979,.T.);
#77175=ORIENTED_EDGE('',*,*,#54980,.T.);
#77176=ORIENTED_EDGE('',*,*,#54981,.T.);
#77177=ORIENTED_EDGE('',*,*,#54982,.T.);
#77178=ORIENTED_EDGE('',*,*,#54983,.T.);
#77179=ORIENTED_EDGE('',*,*,#54984,.T.);
#77180=ORIENTED_EDGE('',*,*,#54985,.T.);
#77181=ORIENTED_EDGE('',*,*,#54986,.T.);
#77182=ORIENTED_EDGE('',*,*,#54987,.T.);
#77183=ORIENTED_EDGE('',*,*,#54988,.T.);
#77184=ORIENTED_EDGE('',*,*,#54989,.T.);
#77185=ORIENTED_EDGE('',*,*,#54990,.T.);
#77186=ORIENTED_EDGE('',*,*,#54991,.T.);
#77187=ORIENTED_EDGE('',*,*,#54992,.T.);
#77188=ORIENTED_EDGE('',*,*,#54993,.T.);
#77189=ORIENTED_EDGE('',*,*,#54994,.T.);
#77190=ORIENTED_EDGE('',*,*,#54995,.T.);
#77191=ORIENTED_EDGE('',*,*,#54996,.T.);
#77192=ORIENTED_EDGE('',*,*,#54997,.T.);
#77193=ORIENTED_EDGE('',*,*,#54998,.T.);
#77194=ORIENTED_EDGE('',*,*,#54999,.T.);
#77195=ORIENTED_EDGE('',*,*,#55000,.T.);
#77196=ORIENTED_EDGE('',*,*,#55001,.T.);
#77197=ORIENTED_EDGE('',*,*,#55002,.T.);
#77198=ORIENTED_EDGE('',*,*,#55003,.T.);
#77199=ORIENTED_EDGE('',*,*,#55004,.T.);
#77200=ORIENTED_EDGE('',*,*,#55005,.T.);
#77201=ORIENTED_EDGE('',*,*,#55006,.T.);
#77202=ORIENTED_EDGE('',*,*,#55007,.T.);
#77203=ORIENTED_EDGE('',*,*,#55008,.T.);
#77204=ORIENTED_EDGE('',*,*,#55009,.T.);
#77205=ORIENTED_EDGE('',*,*,#55010,.T.);
#77206=ORIENTED_EDGE('',*,*,#55011,.T.);
#77207=ORIENTED_EDGE('',*,*,#55012,.T.);
#77208=ORIENTED_EDGE('',*,*,#55013,.T.);
#77209=ORIENTED_EDGE('',*,*,#55014,.T.);
#77210=ORIENTED_EDGE('',*,*,#55015,.T.);
#77211=ORIENTED_EDGE('',*,*,#55016,.T.);
#77212=ORIENTED_EDGE('',*,*,#55017,.T.);
#77213=ORIENTED_EDGE('',*,*,#55018,.T.);
#77214=ORIENTED_EDGE('',*,*,#55019,.T.);
#77215=ORIENTED_EDGE('',*,*,#55020,.T.);
#77216=ORIENTED_EDGE('',*,*,#55021,.T.);
#77217=ORIENTED_EDGE('',*,*,#55022,.T.);
#77218=ORIENTED_EDGE('',*,*,#55023,.T.);
#77219=ORIENTED_EDGE('',*,*,#55024,.T.);
#77220=ORIENTED_EDGE('',*,*,#55025,.T.);
#77221=ORIENTED_EDGE('',*,*,#55026,.T.);
#77222=ORIENTED_EDGE('',*,*,#55027,.T.);
#77223=ORIENTED_EDGE('',*,*,#55028,.T.);
#77224=ORIENTED_EDGE('',*,*,#55029,.T.);
#77225=ORIENTED_EDGE('',*,*,#55030,.T.);
#77226=ORIENTED_EDGE('',*,*,#55031,.T.);
#77227=ORIENTED_EDGE('',*,*,#55032,.T.);
#77228=ORIENTED_EDGE('',*,*,#55033,.T.);
#77229=ORIENTED_EDGE('',*,*,#55034,.T.);
#77230=ORIENTED_EDGE('',*,*,#55035,.T.);
#77231=ORIENTED_EDGE('',*,*,#55036,.T.);
#77232=ORIENTED_EDGE('',*,*,#55037,.T.);
#77233=ORIENTED_EDGE('',*,*,#55038,.T.);
#77234=ORIENTED_EDGE('',*,*,#55039,.T.);
#77235=ORIENTED_EDGE('',*,*,#55040,.T.);
#77236=ORIENTED_EDGE('',*,*,#55041,.T.);
#77237=ORIENTED_EDGE('',*,*,#55042,.T.);
#77238=ORIENTED_EDGE('',*,*,#55043,.T.);
#77239=ORIENTED_EDGE('',*,*,#55044,.T.);
#77240=ORIENTED_EDGE('',*,*,#55045,.T.);
#77241=ORIENTED_EDGE('',*,*,#55046,.T.);
#77242=ORIENTED_EDGE('',*,*,#55047,.T.);
#77243=ORIENTED_EDGE('',*,*,#55048,.T.);
#77244=ORIENTED_EDGE('',*,*,#55049,.T.);
#77245=ORIENTED_EDGE('',*,*,#55050,.T.);
#77246=ORIENTED_EDGE('',*,*,#55051,.T.);
#77247=ORIENTED_EDGE('',*,*,#55052,.T.);
#77248=ORIENTED_EDGE('',*,*,#55053,.T.);
#77249=ORIENTED_EDGE('',*,*,#55054,.T.);
#77250=ORIENTED_EDGE('',*,*,#55055,.T.);
#77251=ORIENTED_EDGE('',*,*,#55056,.T.);
#77252=ORIENTED_EDGE('',*,*,#55057,.T.);
#77253=ORIENTED_EDGE('',*,*,#55058,.T.);
#77254=ORIENTED_EDGE('',*,*,#55059,.T.);
#77255=ORIENTED_EDGE('',*,*,#55060,.T.);
#77256=ORIENTED_EDGE('',*,*,#55061,.T.);
#77257=ORIENTED_EDGE('',*,*,#55062,.T.);
#77258=ORIENTED_EDGE('',*,*,#55063,.T.);
#77259=ORIENTED_EDGE('',*,*,#55064,.T.);
#77260=ORIENTED_EDGE('',*,*,#55065,.T.);
#77261=ORIENTED_EDGE('',*,*,#55066,.T.);
#77262=ORIENTED_EDGE('',*,*,#55067,.T.);
#77263=ORIENTED_EDGE('',*,*,#55068,.T.);
#77264=ORIENTED_EDGE('',*,*,#55069,.T.);
#77265=ORIENTED_EDGE('',*,*,#55070,.T.);
#77266=ORIENTED_EDGE('',*,*,#55071,.T.);
#77267=ORIENTED_EDGE('',*,*,#55072,.T.);
#77268=ORIENTED_EDGE('',*,*,#55073,.T.);
#77269=ORIENTED_EDGE('',*,*,#55074,.T.);
#77270=ORIENTED_EDGE('',*,*,#55075,.T.);
#77271=ORIENTED_EDGE('',*,*,#55076,.T.);
#77272=ORIENTED_EDGE('',*,*,#55077,.T.);
#77273=ORIENTED_EDGE('',*,*,#55078,.T.);
#77274=ORIENTED_EDGE('',*,*,#55079,.T.);
#77275=ORIENTED_EDGE('',*,*,#55080,.T.);
#77276=ORIENTED_EDGE('',*,*,#55081,.T.);
#77277=ORIENTED_EDGE('',*,*,#55082,.T.);
#77278=ORIENTED_EDGE('',*,*,#55083,.T.);
#77279=ORIENTED_EDGE('',*,*,#55084,.T.);
#77280=ORIENTED_EDGE('',*,*,#55085,.T.);
#77281=ORIENTED_EDGE('',*,*,#55086,.T.);
#77282=ORIENTED_EDGE('',*,*,#55087,.T.);
#77283=ORIENTED_EDGE('',*,*,#55088,.T.);
#77284=ORIENTED_EDGE('',*,*,#55089,.T.);
#77285=ORIENTED_EDGE('',*,*,#55090,.T.);
#77286=ORIENTED_EDGE('',*,*,#55091,.T.);
#77287=ORIENTED_EDGE('',*,*,#55092,.T.);
#77288=ORIENTED_EDGE('',*,*,#55093,.T.);
#77289=ORIENTED_EDGE('',*,*,#55094,.T.);
#77290=ORIENTED_EDGE('',*,*,#55095,.T.);
#77291=ORIENTED_EDGE('',*,*,#55096,.T.);
#77292=ORIENTED_EDGE('',*,*,#55097,.T.);
#77293=ORIENTED_EDGE('',*,*,#55098,.T.);
#77294=ORIENTED_EDGE('',*,*,#55099,.T.);
#77295=ORIENTED_EDGE('',*,*,#55100,.T.);
#77296=ORIENTED_EDGE('',*,*,#55101,.T.);
#77297=ORIENTED_EDGE('',*,*,#55102,.T.);
#77298=ORIENTED_EDGE('',*,*,#55103,.T.);
#77299=ORIENTED_EDGE('',*,*,#55104,.T.);
#77300=ORIENTED_EDGE('',*,*,#55105,.T.);
#77301=ORIENTED_EDGE('',*,*,#55106,.T.);
#77302=ORIENTED_EDGE('',*,*,#55107,.T.);
#77303=ORIENTED_EDGE('',*,*,#55108,.T.);
#77304=ORIENTED_EDGE('',*,*,#55109,.T.);
#77305=ORIENTED_EDGE('',*,*,#55110,.T.);
#77306=ORIENTED_EDGE('',*,*,#55111,.T.);
#77307=ORIENTED_EDGE('',*,*,#55112,.T.);
#77308=ORIENTED_EDGE('',*,*,#55113,.T.);
#77309=ORIENTED_EDGE('',*,*,#55114,.T.);
#77310=ORIENTED_EDGE('',*,*,#55115,.T.);
#77311=ORIENTED_EDGE('',*,*,#55116,.T.);
#77312=ORIENTED_EDGE('',*,*,#55117,.T.);
#77313=ORIENTED_EDGE('',*,*,#55118,.T.);
#77314=ORIENTED_EDGE('',*,*,#55119,.T.);
#77315=ORIENTED_EDGE('',*,*,#55120,.T.);
#77316=ORIENTED_EDGE('',*,*,#55121,.T.);
#77317=ORIENTED_EDGE('',*,*,#55122,.T.);
#77318=ORIENTED_EDGE('',*,*,#55123,.T.);
#77319=ORIENTED_EDGE('',*,*,#55124,.T.);
#77320=ORIENTED_EDGE('',*,*,#55125,.T.);
#77321=ORIENTED_EDGE('',*,*,#55126,.T.);
#77322=ORIENTED_EDGE('',*,*,#55127,.T.);
#77323=ORIENTED_EDGE('',*,*,#55128,.T.);
#77324=ORIENTED_EDGE('',*,*,#55129,.T.);
#77325=ORIENTED_EDGE('',*,*,#55130,.T.);
#77326=ORIENTED_EDGE('',*,*,#55131,.T.);
#77327=ORIENTED_EDGE('',*,*,#55132,.T.);
#77328=ORIENTED_EDGE('',*,*,#55133,.T.);
#77329=ORIENTED_EDGE('',*,*,#55134,.T.);
#77330=ORIENTED_EDGE('',*,*,#55135,.T.);
#77331=ORIENTED_EDGE('',*,*,#55136,.T.);
#77332=ORIENTED_EDGE('',*,*,#55137,.T.);
#77333=ORIENTED_EDGE('',*,*,#55138,.T.);
#77334=ORIENTED_EDGE('',*,*,#55139,.T.);
#77335=ORIENTED_EDGE('',*,*,#55140,.T.);
#77336=ORIENTED_EDGE('',*,*,#55141,.T.);
#77337=ORIENTED_EDGE('',*,*,#55142,.T.);
#77338=ORIENTED_EDGE('',*,*,#55143,.T.);
#77339=ORIENTED_EDGE('',*,*,#55144,.T.);
#77340=ORIENTED_EDGE('',*,*,#55145,.T.);
#77341=ORIENTED_EDGE('',*,*,#55146,.T.);
#77342=ORIENTED_EDGE('',*,*,#55147,.T.);
#77343=ORIENTED_EDGE('',*,*,#55148,.T.);
#77344=ORIENTED_EDGE('',*,*,#55149,.T.);
#77345=ORIENTED_EDGE('',*,*,#55150,.T.);
#77346=ORIENTED_EDGE('',*,*,#55151,.T.);
#77347=ORIENTED_EDGE('',*,*,#55152,.T.);
#77348=ORIENTED_EDGE('',*,*,#55153,.T.);
#77349=ORIENTED_EDGE('',*,*,#55154,.T.);
#77350=ORIENTED_EDGE('',*,*,#55155,.T.);
#77351=ORIENTED_EDGE('',*,*,#55156,.T.);
#77352=ORIENTED_EDGE('',*,*,#55157,.T.);
#77353=ORIENTED_EDGE('',*,*,#55158,.T.);
#77354=ORIENTED_EDGE('',*,*,#55159,.T.);
#77355=ORIENTED_EDGE('',*,*,#55160,.T.);
#77356=ORIENTED_EDGE('',*,*,#55161,.T.);
#77357=ORIENTED_EDGE('',*,*,#55162,.T.);
#77358=ORIENTED_EDGE('',*,*,#55163,.T.);
#77359=ORIENTED_EDGE('',*,*,#55164,.T.);
#77360=ORIENTED_EDGE('',*,*,#55165,.T.);
#77361=ORIENTED_EDGE('',*,*,#55166,.T.);
#77362=ORIENTED_EDGE('',*,*,#55167,.T.);
#77363=ORIENTED_EDGE('',*,*,#55168,.T.);
#77364=ORIENTED_EDGE('',*,*,#55169,.T.);
#77365=ORIENTED_EDGE('',*,*,#55170,.T.);
#77366=ORIENTED_EDGE('',*,*,#55171,.T.);
#77367=ORIENTED_EDGE('',*,*,#55172,.T.);
#77368=ORIENTED_EDGE('',*,*,#55173,.T.);
#77369=ORIENTED_EDGE('',*,*,#55174,.T.);
#77370=ORIENTED_EDGE('',*,*,#55175,.T.);
#77371=ORIENTED_EDGE('',*,*,#55176,.T.);
#77372=ORIENTED_EDGE('',*,*,#55177,.T.);
#77373=ORIENTED_EDGE('',*,*,#55178,.T.);
#77374=ORIENTED_EDGE('',*,*,#55179,.T.);
#77375=ORIENTED_EDGE('',*,*,#55180,.T.);
#77376=ORIENTED_EDGE('',*,*,#55181,.T.);
#77377=ORIENTED_EDGE('',*,*,#55182,.T.);
#77378=ORIENTED_EDGE('',*,*,#55183,.T.);
#77379=ORIENTED_EDGE('',*,*,#55184,.T.);
#77380=ORIENTED_EDGE('',*,*,#55185,.T.);
#77381=ORIENTED_EDGE('',*,*,#55186,.T.);
#77382=ORIENTED_EDGE('',*,*,#55187,.T.);
#77383=ORIENTED_EDGE('',*,*,#55188,.T.);
#77384=ORIENTED_EDGE('',*,*,#55189,.T.);
#77385=ORIENTED_EDGE('',*,*,#55190,.T.);
#77386=ORIENTED_EDGE('',*,*,#55191,.T.);
#77387=ORIENTED_EDGE('',*,*,#55192,.T.);
#77388=ORIENTED_EDGE('',*,*,#55193,.T.);
#77389=ORIENTED_EDGE('',*,*,#55194,.T.);
#77390=ORIENTED_EDGE('',*,*,#55195,.T.);
#77391=ORIENTED_EDGE('',*,*,#55196,.T.);
#77392=ORIENTED_EDGE('',*,*,#55197,.T.);
#77393=ORIENTED_EDGE('',*,*,#55198,.T.);
#77394=ORIENTED_EDGE('',*,*,#55199,.T.);
#77395=ORIENTED_EDGE('',*,*,#55200,.T.);
#77396=ORIENTED_EDGE('',*,*,#55201,.T.);
#77397=ORIENTED_EDGE('',*,*,#55202,.T.);
#77398=ORIENTED_EDGE('',*,*,#55203,.T.);
#77399=ORIENTED_EDGE('',*,*,#55204,.T.);
#77400=ORIENTED_EDGE('',*,*,#55205,.T.);
#77401=ORIENTED_EDGE('',*,*,#55206,.T.);
#77402=ORIENTED_EDGE('',*,*,#55207,.T.);
#77403=ORIENTED_EDGE('',*,*,#55208,.T.);
#77404=ORIENTED_EDGE('',*,*,#55209,.T.);
#77405=ORIENTED_EDGE('',*,*,#55210,.T.);
#77406=ORIENTED_EDGE('',*,*,#55211,.T.);
#77407=ORIENTED_EDGE('',*,*,#55212,.T.);
#77408=ORIENTED_EDGE('',*,*,#55213,.T.);
#77409=ORIENTED_EDGE('',*,*,#55214,.T.);
#77410=ORIENTED_EDGE('',*,*,#55215,.T.);
#77411=ORIENTED_EDGE('',*,*,#55216,.T.);
#77412=ORIENTED_EDGE('',*,*,#55217,.T.);
#77413=ORIENTED_EDGE('',*,*,#55218,.T.);
#77414=ORIENTED_EDGE('',*,*,#55219,.T.);
#77415=ORIENTED_EDGE('',*,*,#55220,.T.);
#77416=ORIENTED_EDGE('',*,*,#55221,.T.);
#77417=ORIENTED_EDGE('',*,*,#55222,.T.);
#77418=ORIENTED_EDGE('',*,*,#55223,.T.);
#77419=ORIENTED_EDGE('',*,*,#55224,.T.);
#77420=ORIENTED_EDGE('',*,*,#55225,.T.);
#77421=ORIENTED_EDGE('',*,*,#55226,.T.);
#77422=ORIENTED_EDGE('',*,*,#55227,.T.);
#77423=ORIENTED_EDGE('',*,*,#55228,.T.);
#77424=ORIENTED_EDGE('',*,*,#55229,.T.);
#77425=ORIENTED_EDGE('',*,*,#55230,.T.);
#77426=ORIENTED_EDGE('',*,*,#55231,.T.);
#77427=ORIENTED_EDGE('',*,*,#55232,.T.);
#77428=ORIENTED_EDGE('',*,*,#55233,.T.);
#77429=ORIENTED_EDGE('',*,*,#55234,.T.);
#77430=ORIENTED_EDGE('',*,*,#55235,.T.);
#77431=ORIENTED_EDGE('',*,*,#55236,.T.);
#77432=ORIENTED_EDGE('',*,*,#55237,.T.);
#77433=ORIENTED_EDGE('',*,*,#55238,.T.);
#77434=ORIENTED_EDGE('',*,*,#55239,.T.);
#77435=ORIENTED_EDGE('',*,*,#55240,.T.);
#77436=ORIENTED_EDGE('',*,*,#55241,.T.);
#77437=ORIENTED_EDGE('',*,*,#55242,.T.);
#77438=ORIENTED_EDGE('',*,*,#55243,.T.);
#77439=ORIENTED_EDGE('',*,*,#55244,.T.);
#77440=ORIENTED_EDGE('',*,*,#55245,.T.);
#77441=ORIENTED_EDGE('',*,*,#55246,.T.);
#77442=ORIENTED_EDGE('',*,*,#55247,.T.);
#77443=ORIENTED_EDGE('',*,*,#55248,.T.);
#77444=ORIENTED_EDGE('',*,*,#55249,.T.);
#77445=ORIENTED_EDGE('',*,*,#55250,.T.);
#77446=ORIENTED_EDGE('',*,*,#55251,.T.);
#77447=ORIENTED_EDGE('',*,*,#55252,.T.);
#77448=ORIENTED_EDGE('',*,*,#55253,.T.);
#77449=ORIENTED_EDGE('',*,*,#55254,.T.);
#77450=ORIENTED_EDGE('',*,*,#55255,.T.);
#77451=ORIENTED_EDGE('',*,*,#55256,.T.);
#77452=ORIENTED_EDGE('',*,*,#55257,.T.);
#77453=ORIENTED_EDGE('',*,*,#55258,.T.);
#77454=ORIENTED_EDGE('',*,*,#55259,.T.);
#77455=ORIENTED_EDGE('',*,*,#55260,.T.);
#77456=ORIENTED_EDGE('',*,*,#55261,.T.);
#77457=ORIENTED_EDGE('',*,*,#55262,.T.);
#77458=ORIENTED_EDGE('',*,*,#55263,.T.);
#77459=ORIENTED_EDGE('',*,*,#55264,.T.);
#77460=ORIENTED_EDGE('',*,*,#55265,.T.);
#77461=ORIENTED_EDGE('',*,*,#55266,.T.);
#77462=ORIENTED_EDGE('',*,*,#55267,.T.);
#77463=ORIENTED_EDGE('',*,*,#55268,.T.);
#77464=ORIENTED_EDGE('',*,*,#55269,.T.);
#77465=ORIENTED_EDGE('',*,*,#55270,.T.);
#77466=ORIENTED_EDGE('',*,*,#55271,.T.);
#77467=ORIENTED_EDGE('',*,*,#55272,.T.);
#77468=ORIENTED_EDGE('',*,*,#55273,.T.);
#77469=ORIENTED_EDGE('',*,*,#55274,.T.);
#77470=ORIENTED_EDGE('',*,*,#55275,.T.);
#77471=ORIENTED_EDGE('',*,*,#55276,.T.);
#77472=ORIENTED_EDGE('',*,*,#55277,.T.);
#77473=ORIENTED_EDGE('',*,*,#55278,.T.);
#77474=ORIENTED_EDGE('',*,*,#55279,.T.);
#77475=ORIENTED_EDGE('',*,*,#55280,.T.);
#77476=ORIENTED_EDGE('',*,*,#55281,.T.);
#77477=ORIENTED_EDGE('',*,*,#55282,.T.);
#77478=ORIENTED_EDGE('',*,*,#55283,.T.);
#77479=ORIENTED_EDGE('',*,*,#55284,.T.);
#77480=ORIENTED_EDGE('',*,*,#55285,.T.);
#77481=ORIENTED_EDGE('',*,*,#55286,.T.);
#77482=ORIENTED_EDGE('',*,*,#55287,.T.);
#77483=ORIENTED_EDGE('',*,*,#55288,.T.);
#77484=ORIENTED_EDGE('',*,*,#55289,.T.);
#77485=ORIENTED_EDGE('',*,*,#55290,.T.);
#77486=ORIENTED_EDGE('',*,*,#55291,.T.);
#77487=ORIENTED_EDGE('',*,*,#55292,.T.);
#77488=ORIENTED_EDGE('',*,*,#55293,.T.);
#77489=ORIENTED_EDGE('',*,*,#55294,.T.);
#77490=ORIENTED_EDGE('',*,*,#55295,.T.);
#77491=ORIENTED_EDGE('',*,*,#55296,.T.);
#77492=ORIENTED_EDGE('',*,*,#55297,.T.);
#77493=ORIENTED_EDGE('',*,*,#55298,.T.);
#77494=ORIENTED_EDGE('',*,*,#55299,.T.);
#77495=ORIENTED_EDGE('',*,*,#55300,.T.);
#77496=ORIENTED_EDGE('',*,*,#55301,.T.);
#77497=ORIENTED_EDGE('',*,*,#55302,.T.);
#77498=ORIENTED_EDGE('',*,*,#55303,.T.);
#77499=ORIENTED_EDGE('',*,*,#55304,.T.);
#77500=ORIENTED_EDGE('',*,*,#55305,.T.);
#77501=ORIENTED_EDGE('',*,*,#55306,.T.);
#77502=ORIENTED_EDGE('',*,*,#55307,.T.);
#77503=ORIENTED_EDGE('',*,*,#55308,.T.);
#77504=ORIENTED_EDGE('',*,*,#55309,.T.);
#77505=ORIENTED_EDGE('',*,*,#55310,.T.);
#77506=ORIENTED_EDGE('',*,*,#55311,.T.);
#77507=ORIENTED_EDGE('',*,*,#55312,.T.);
#77508=ORIENTED_EDGE('',*,*,#55313,.T.);
#77509=ORIENTED_EDGE('',*,*,#55314,.T.);
#77510=ORIENTED_EDGE('',*,*,#55315,.T.);
#77511=ORIENTED_EDGE('',*,*,#55316,.T.);
#77512=ORIENTED_EDGE('',*,*,#55317,.T.);
#77513=ORIENTED_EDGE('',*,*,#55318,.T.);
#77514=ORIENTED_EDGE('',*,*,#55319,.T.);
#77515=ORIENTED_EDGE('',*,*,#55320,.T.);
#77516=ORIENTED_EDGE('',*,*,#55321,.T.);
#77517=ORIENTED_EDGE('',*,*,#55322,.T.);
#77518=ORIENTED_EDGE('',*,*,#55323,.T.);
#77519=ORIENTED_EDGE('',*,*,#55324,.T.);
#77520=ORIENTED_EDGE('',*,*,#55325,.T.);
#77521=ORIENTED_EDGE('',*,*,#55326,.T.);
#77522=ORIENTED_EDGE('',*,*,#55327,.T.);
#77523=ORIENTED_EDGE('',*,*,#55328,.T.);
#77524=ORIENTED_EDGE('',*,*,#55329,.T.);
#77525=ORIENTED_EDGE('',*,*,#55330,.T.);
#77526=ORIENTED_EDGE('',*,*,#55331,.T.);
#77527=ORIENTED_EDGE('',*,*,#55332,.T.);
#77528=ORIENTED_EDGE('',*,*,#55333,.T.);
#77529=ORIENTED_EDGE('',*,*,#55334,.T.);
#77530=ORIENTED_EDGE('',*,*,#55335,.T.);
#77531=ORIENTED_EDGE('',*,*,#55336,.T.);
#77532=ORIENTED_EDGE('',*,*,#55337,.T.);
#77533=ORIENTED_EDGE('',*,*,#55338,.T.);
#77534=ORIENTED_EDGE('',*,*,#55339,.T.);
#77535=ORIENTED_EDGE('',*,*,#55340,.T.);
#77536=ORIENTED_EDGE('',*,*,#55341,.T.);
#77537=ORIENTED_EDGE('',*,*,#55342,.T.);
#77538=ORIENTED_EDGE('',*,*,#55343,.T.);
#77539=ORIENTED_EDGE('',*,*,#55344,.T.);
#77540=ORIENTED_EDGE('',*,*,#55345,.T.);
#77541=ORIENTED_EDGE('',*,*,#55346,.T.);
#77542=ORIENTED_EDGE('',*,*,#55347,.T.);
#77543=ORIENTED_EDGE('',*,*,#55348,.T.);
#77544=ORIENTED_EDGE('',*,*,#55349,.T.);
#77545=ORIENTED_EDGE('',*,*,#55350,.T.);
#77546=ORIENTED_EDGE('',*,*,#55351,.T.);
#77547=ORIENTED_EDGE('',*,*,#55352,.T.);
#77548=ORIENTED_EDGE('',*,*,#55353,.T.);
#77549=ORIENTED_EDGE('',*,*,#55354,.T.);
#77550=ORIENTED_EDGE('',*,*,#55355,.T.);
#77551=ORIENTED_EDGE('',*,*,#55356,.T.);
#77552=ORIENTED_EDGE('',*,*,#55357,.T.);
#77553=ORIENTED_EDGE('',*,*,#55358,.T.);
#77554=ORIENTED_EDGE('',*,*,#55359,.T.);
#77555=ORIENTED_EDGE('',*,*,#55360,.T.);
#77556=ORIENTED_EDGE('',*,*,#55361,.T.);
#77557=ORIENTED_EDGE('',*,*,#55362,.T.);
#77558=ORIENTED_EDGE('',*,*,#55363,.T.);
#77559=ORIENTED_EDGE('',*,*,#55364,.T.);
#77560=ORIENTED_EDGE('',*,*,#55365,.T.);
#77561=ORIENTED_EDGE('',*,*,#55366,.T.);
#77562=ORIENTED_EDGE('',*,*,#55367,.T.);
#77563=ORIENTED_EDGE('',*,*,#55368,.T.);
#77564=ORIENTED_EDGE('',*,*,#55369,.T.);
#77565=ORIENTED_EDGE('',*,*,#55370,.T.);
#77566=ORIENTED_EDGE('',*,*,#55371,.T.);
#77567=ORIENTED_EDGE('',*,*,#55372,.T.);
#77568=ORIENTED_EDGE('',*,*,#55373,.T.);
#77569=ORIENTED_EDGE('',*,*,#55374,.T.);
#77570=ORIENTED_EDGE('',*,*,#55375,.T.);
#77571=ORIENTED_EDGE('',*,*,#55376,.T.);
#77572=ORIENTED_EDGE('',*,*,#55377,.T.);
#77573=ORIENTED_EDGE('',*,*,#55378,.T.);
#77574=ORIENTED_EDGE('',*,*,#55379,.T.);
#77575=ORIENTED_EDGE('',*,*,#55380,.T.);
#77576=ORIENTED_EDGE('',*,*,#55381,.T.);
#77577=ORIENTED_EDGE('',*,*,#55382,.T.);
#77578=ORIENTED_EDGE('',*,*,#55383,.T.);
#77579=ORIENTED_EDGE('',*,*,#55384,.T.);
#77580=ORIENTED_EDGE('',*,*,#55385,.T.);
#77581=ORIENTED_EDGE('',*,*,#55386,.T.);
#77582=ORIENTED_EDGE('',*,*,#55387,.T.);
#77583=ORIENTED_EDGE('',*,*,#55388,.T.);
#77584=ORIENTED_EDGE('',*,*,#55389,.T.);
#77585=ORIENTED_EDGE('',*,*,#55390,.T.);
#77586=ORIENTED_EDGE('',*,*,#55391,.T.);
#77587=ORIENTED_EDGE('',*,*,#55392,.T.);
#77588=ORIENTED_EDGE('',*,*,#55393,.T.);
#77589=ORIENTED_EDGE('',*,*,#55394,.T.);
#77590=ORIENTED_EDGE('',*,*,#55395,.T.);
#77591=ORIENTED_EDGE('',*,*,#55396,.T.);
#77592=ORIENTED_EDGE('',*,*,#55397,.T.);
#77593=ORIENTED_EDGE('',*,*,#55398,.T.);
#77594=ORIENTED_EDGE('',*,*,#55399,.T.);
#77595=ORIENTED_EDGE('',*,*,#55400,.T.);
#77596=ORIENTED_EDGE('',*,*,#55401,.T.);
#77597=ORIENTED_EDGE('',*,*,#55402,.T.);
#77598=ORIENTED_EDGE('',*,*,#55403,.T.);
#77599=ORIENTED_EDGE('',*,*,#55404,.T.);
#77600=ORIENTED_EDGE('',*,*,#55405,.T.);
#77601=ORIENTED_EDGE('',*,*,#55406,.T.);
#77602=ORIENTED_EDGE('',*,*,#55407,.T.);
#77603=ORIENTED_EDGE('',*,*,#55408,.T.);
#77604=ORIENTED_EDGE('',*,*,#55409,.T.);
#77605=ORIENTED_EDGE('',*,*,#55410,.T.);
#77606=ORIENTED_EDGE('',*,*,#55411,.T.);
#77607=ORIENTED_EDGE('',*,*,#55412,.T.);
#77608=ORIENTED_EDGE('',*,*,#55413,.T.);
#77609=ORIENTED_EDGE('',*,*,#55414,.T.);
#77610=ORIENTED_EDGE('',*,*,#55415,.T.);
#77611=ORIENTED_EDGE('',*,*,#55416,.T.);
#77612=ORIENTED_EDGE('',*,*,#55417,.T.);
#77613=ORIENTED_EDGE('',*,*,#55418,.T.);
#77614=ORIENTED_EDGE('',*,*,#55419,.T.);
#77615=ORIENTED_EDGE('',*,*,#55420,.T.);
#77616=ORIENTED_EDGE('',*,*,#55421,.T.);
#77617=ORIENTED_EDGE('',*,*,#55422,.T.);
#77618=ORIENTED_EDGE('',*,*,#55423,.T.);
#77619=ORIENTED_EDGE('',*,*,#55424,.T.);
#77620=ORIENTED_EDGE('',*,*,#55425,.T.);
#77621=ORIENTED_EDGE('',*,*,#55426,.T.);
#77622=ORIENTED_EDGE('',*,*,#55427,.T.);
#77623=ORIENTED_EDGE('',*,*,#55428,.T.);
#77624=ORIENTED_EDGE('',*,*,#55429,.T.);
#77625=ORIENTED_EDGE('',*,*,#55430,.T.);
#77626=ORIENTED_EDGE('',*,*,#55431,.T.);
#77627=ORIENTED_EDGE('',*,*,#55432,.T.);
#77628=ORIENTED_EDGE('',*,*,#55433,.T.);
#77629=ORIENTED_EDGE('',*,*,#55434,.T.);
#77630=ORIENTED_EDGE('',*,*,#55435,.T.);
#77631=ORIENTED_EDGE('',*,*,#55436,.T.);
#77632=ORIENTED_EDGE('',*,*,#55437,.T.);
#77633=ORIENTED_EDGE('',*,*,#55438,.T.);
#77634=ORIENTED_EDGE('',*,*,#55439,.T.);
#77635=ORIENTED_EDGE('',*,*,#55440,.T.);
#77636=ORIENTED_EDGE('',*,*,#55441,.T.);
#77637=ORIENTED_EDGE('',*,*,#55442,.T.);
#77638=ORIENTED_EDGE('',*,*,#55443,.T.);
#77639=ORIENTED_EDGE('',*,*,#55444,.T.);
#77640=ORIENTED_EDGE('',*,*,#55445,.T.);
#77641=ORIENTED_EDGE('',*,*,#55446,.T.);
#77642=ORIENTED_EDGE('',*,*,#55447,.T.);
#77643=ORIENTED_EDGE('',*,*,#55448,.T.);
#77644=ORIENTED_EDGE('',*,*,#55449,.T.);
#77645=ORIENTED_EDGE('',*,*,#55450,.T.);
#77646=ORIENTED_EDGE('',*,*,#55451,.T.);
#77647=ORIENTED_EDGE('',*,*,#55452,.T.);
#77648=ORIENTED_EDGE('',*,*,#55453,.T.);
#77649=ORIENTED_EDGE('',*,*,#55454,.T.);
#77650=ORIENTED_EDGE('',*,*,#55455,.T.);
#77651=ORIENTED_EDGE('',*,*,#55456,.T.);
#77652=ORIENTED_EDGE('',*,*,#55457,.T.);
#77653=ORIENTED_EDGE('',*,*,#55458,.T.);
#77654=ORIENTED_EDGE('',*,*,#55459,.T.);
#77655=ORIENTED_EDGE('',*,*,#55460,.T.);
#77656=ORIENTED_EDGE('',*,*,#52043,.T.);
#77657=ORIENTED_EDGE('',*,*,#55461,.T.);
#77658=ORIENTED_EDGE('',*,*,#52037,.T.);
#77659=ORIENTED_EDGE('',*,*,#55462,.T.);
#77660=ORIENTED_EDGE('',*,*,#55463,.T.);
#77661=ORIENTED_EDGE('',*,*,#55464,.T.);
#77662=ORIENTED_EDGE('',*,*,#55465,.T.);
#77663=ORIENTED_EDGE('',*,*,#55466,.T.);
#77664=ORIENTED_EDGE('',*,*,#55467,.T.);
#77665=ORIENTED_EDGE('',*,*,#55468,.T.);
#77666=ORIENTED_EDGE('',*,*,#55469,.T.);
#77667=ORIENTED_EDGE('',*,*,#55470,.T.);
#77668=ORIENTED_EDGE('',*,*,#55471,.T.);
#77669=ORIENTED_EDGE('',*,*,#55472,.T.);
#77670=ORIENTED_EDGE('',*,*,#55473,.T.);
#77671=ORIENTED_EDGE('',*,*,#55474,.T.);
#77672=ORIENTED_EDGE('',*,*,#55475,.T.);
#77673=ORIENTED_EDGE('',*,*,#55476,.T.);
#77674=ORIENTED_EDGE('',*,*,#55477,.T.);
#77675=ORIENTED_EDGE('',*,*,#55478,.T.);
#77676=ORIENTED_EDGE('',*,*,#55479,.T.);
#77677=ORIENTED_EDGE('',*,*,#55480,.T.);
#77678=ORIENTED_EDGE('',*,*,#55481,.T.);
#77679=ORIENTED_EDGE('',*,*,#55482,.T.);
#77680=ORIENTED_EDGE('',*,*,#55483,.T.);
#77681=ORIENTED_EDGE('',*,*,#55484,.T.);
#77682=ORIENTED_EDGE('',*,*,#55485,.T.);
#77683=ORIENTED_EDGE('',*,*,#55486,.T.);
#77684=ORIENTED_EDGE('',*,*,#55487,.T.);
#77685=ORIENTED_EDGE('',*,*,#55488,.T.);
#77686=ORIENTED_EDGE('',*,*,#55489,.T.);
#77687=ORIENTED_EDGE('',*,*,#55490,.T.);
#77688=ORIENTED_EDGE('',*,*,#55491,.T.);
#77689=ORIENTED_EDGE('',*,*,#55492,.T.);
#77690=ORIENTED_EDGE('',*,*,#55493,.T.);
#77691=ORIENTED_EDGE('',*,*,#55494,.T.);
#77692=ORIENTED_EDGE('',*,*,#55495,.T.);
#77693=ORIENTED_EDGE('',*,*,#55496,.T.);
#77694=ORIENTED_EDGE('',*,*,#55497,.T.);
#77695=ORIENTED_EDGE('',*,*,#55498,.T.);
#77696=ORIENTED_EDGE('',*,*,#55499,.T.);
#77697=ORIENTED_EDGE('',*,*,#55500,.T.);
#77698=ORIENTED_EDGE('',*,*,#55501,.T.);
#77699=ORIENTED_EDGE('',*,*,#55502,.T.);
#77700=ORIENTED_EDGE('',*,*,#55503,.T.);
#77701=ORIENTED_EDGE('',*,*,#55504,.T.);
#77702=ORIENTED_EDGE('',*,*,#55505,.T.);
#77703=ORIENTED_EDGE('',*,*,#55506,.T.);
#77704=ORIENTED_EDGE('',*,*,#55507,.T.);
#77705=ORIENTED_EDGE('',*,*,#55508,.T.);
#77706=ORIENTED_EDGE('',*,*,#55509,.T.);
#77707=ORIENTED_EDGE('',*,*,#55510,.T.);
#77708=ORIENTED_EDGE('',*,*,#55511,.T.);
#77709=ORIENTED_EDGE('',*,*,#55512,.T.);
#77710=ORIENTED_EDGE('',*,*,#55513,.T.);
#77711=ORIENTED_EDGE('',*,*,#55514,.T.);
#77712=ORIENTED_EDGE('',*,*,#55515,.T.);
#77713=ORIENTED_EDGE('',*,*,#55516,.T.);
#77714=ORIENTED_EDGE('',*,*,#55517,.T.);
#77715=ORIENTED_EDGE('',*,*,#55518,.T.);
#77716=ORIENTED_EDGE('',*,*,#55519,.T.);
#77717=ORIENTED_EDGE('',*,*,#55520,.T.);
#77718=ORIENTED_EDGE('',*,*,#55521,.T.);
#77719=ORIENTED_EDGE('',*,*,#55522,.T.);
#77720=ORIENTED_EDGE('',*,*,#55523,.T.);
#77721=ORIENTED_EDGE('',*,*,#55524,.T.);
#77722=ORIENTED_EDGE('',*,*,#55525,.T.);
#77723=ORIENTED_EDGE('',*,*,#55526,.T.);
#77724=ORIENTED_EDGE('',*,*,#55527,.T.);
#77725=ORIENTED_EDGE('',*,*,#55528,.T.);
#77726=ORIENTED_EDGE('',*,*,#55529,.T.);
#77727=ORIENTED_EDGE('',*,*,#55530,.T.);
#77728=ORIENTED_EDGE('',*,*,#55531,.T.);
#77729=ORIENTED_EDGE('',*,*,#55532,.T.);
#77730=ORIENTED_EDGE('',*,*,#55533,.T.);
#77731=ORIENTED_EDGE('',*,*,#55534,.T.);
#77732=ORIENTED_EDGE('',*,*,#55535,.T.);
#77733=ORIENTED_EDGE('',*,*,#55536,.T.);
#77734=ORIENTED_EDGE('',*,*,#55537,.T.);
#77735=ORIENTED_EDGE('',*,*,#55538,.T.);
#77736=ORIENTED_EDGE('',*,*,#55539,.T.);
#77737=ORIENTED_EDGE('',*,*,#55540,.T.);
#77738=ORIENTED_EDGE('',*,*,#55541,.T.);
#77739=ORIENTED_EDGE('',*,*,#55542,.T.);
#77740=ORIENTED_EDGE('',*,*,#55543,.T.);
#77741=ORIENTED_EDGE('',*,*,#55544,.T.);
#77742=ORIENTED_EDGE('',*,*,#55545,.T.);
#77743=ORIENTED_EDGE('',*,*,#55546,.T.);
#77744=ORIENTED_EDGE('',*,*,#55547,.T.);
#77745=ORIENTED_EDGE('',*,*,#55548,.T.);
#77746=ORIENTED_EDGE('',*,*,#55549,.T.);
#77747=ORIENTED_EDGE('',*,*,#55550,.T.);
#77748=ORIENTED_EDGE('',*,*,#55551,.T.);
#77749=ORIENTED_EDGE('',*,*,#55552,.T.);
#77750=ORIENTED_EDGE('',*,*,#55553,.T.);
#77751=ORIENTED_EDGE('',*,*,#55554,.T.);
#77752=ORIENTED_EDGE('',*,*,#55555,.T.);
#77753=ORIENTED_EDGE('',*,*,#55556,.T.);
#77754=ORIENTED_EDGE('',*,*,#55557,.T.);
#77755=ORIENTED_EDGE('',*,*,#55558,.T.);
#77756=ORIENTED_EDGE('',*,*,#55559,.T.);
#77757=ORIENTED_EDGE('',*,*,#55560,.T.);
#77758=ORIENTED_EDGE('',*,*,#55561,.T.);
#77759=ORIENTED_EDGE('',*,*,#55562,.T.);
#77760=ORIENTED_EDGE('',*,*,#55563,.T.);
#77761=ORIENTED_EDGE('',*,*,#55564,.T.);
#77762=ORIENTED_EDGE('',*,*,#55565,.T.);
#77763=ORIENTED_EDGE('',*,*,#55566,.T.);
#77764=ORIENTED_EDGE('',*,*,#55567,.T.);
#77765=ORIENTED_EDGE('',*,*,#55568,.T.);
#77766=ORIENTED_EDGE('',*,*,#55569,.T.);
#77767=ORIENTED_EDGE('',*,*,#55570,.T.);
#77768=ORIENTED_EDGE('',*,*,#55571,.T.);
#77769=ORIENTED_EDGE('',*,*,#55572,.T.);
#77770=ORIENTED_EDGE('',*,*,#55573,.T.);
#77771=ORIENTED_EDGE('',*,*,#55574,.T.);
#77772=ORIENTED_EDGE('',*,*,#55575,.T.);
#77773=ORIENTED_EDGE('',*,*,#55576,.T.);
#77774=ORIENTED_EDGE('',*,*,#55577,.T.);
#77775=ORIENTED_EDGE('',*,*,#55578,.T.);
#77776=ORIENTED_EDGE('',*,*,#55579,.T.);
#77777=ORIENTED_EDGE('',*,*,#55580,.T.);
#77778=ORIENTED_EDGE('',*,*,#55581,.T.);
#77779=ORIENTED_EDGE('',*,*,#55582,.T.);
#77780=ORIENTED_EDGE('',*,*,#55583,.T.);
#77781=ORIENTED_EDGE('',*,*,#55584,.T.);
#77782=ORIENTED_EDGE('',*,*,#55585,.T.);
#77783=ORIENTED_EDGE('',*,*,#55586,.T.);
#77784=ORIENTED_EDGE('',*,*,#55587,.T.);
#77785=ORIENTED_EDGE('',*,*,#55588,.T.);
#77786=ORIENTED_EDGE('',*,*,#55589,.T.);
#77787=ORIENTED_EDGE('',*,*,#55590,.T.);
#77788=ORIENTED_EDGE('',*,*,#55591,.T.);
#77789=ORIENTED_EDGE('',*,*,#55592,.T.);
#77790=ORIENTED_EDGE('',*,*,#55593,.T.);
#77791=ORIENTED_EDGE('',*,*,#55594,.T.);
#77792=ORIENTED_EDGE('',*,*,#55595,.T.);
#77793=ORIENTED_EDGE('',*,*,#55596,.T.);
#77794=ORIENTED_EDGE('',*,*,#55597,.T.);
#77795=ORIENTED_EDGE('',*,*,#55598,.T.);
#77796=ORIENTED_EDGE('',*,*,#55599,.T.);
#77797=ORIENTED_EDGE('',*,*,#55600,.T.);
#77798=ORIENTED_EDGE('',*,*,#55601,.T.);
#77799=ORIENTED_EDGE('',*,*,#55602,.T.);
#77800=ORIENTED_EDGE('',*,*,#55603,.T.);
#77801=ORIENTED_EDGE('',*,*,#55604,.T.);
#77802=ORIENTED_EDGE('',*,*,#55605,.T.);
#77803=ORIENTED_EDGE('',*,*,#55606,.T.);
#77804=ORIENTED_EDGE('',*,*,#55607,.T.);
#77805=ORIENTED_EDGE('',*,*,#55608,.T.);
#77806=ORIENTED_EDGE('',*,*,#55609,.T.);
#77807=ORIENTED_EDGE('',*,*,#55610,.T.);
#77808=ORIENTED_EDGE('',*,*,#55611,.T.);
#77809=ORIENTED_EDGE('',*,*,#55612,.T.);
#77810=ORIENTED_EDGE('',*,*,#55613,.T.);
#77811=ORIENTED_EDGE('',*,*,#55614,.T.);
#77812=ORIENTED_EDGE('',*,*,#55615,.T.);
#77813=ORIENTED_EDGE('',*,*,#55616,.T.);
#77814=ORIENTED_EDGE('',*,*,#55617,.T.);
#77815=ORIENTED_EDGE('',*,*,#55618,.T.);
#77816=ORIENTED_EDGE('',*,*,#55619,.T.);
#77817=ORIENTED_EDGE('',*,*,#55620,.T.);
#77818=ORIENTED_EDGE('',*,*,#55621,.T.);
#77819=ORIENTED_EDGE('',*,*,#55622,.T.);
#77820=ORIENTED_EDGE('',*,*,#55623,.T.);
#77821=ORIENTED_EDGE('',*,*,#55624,.T.);
#77822=ORIENTED_EDGE('',*,*,#55625,.T.);
#77823=ORIENTED_EDGE('',*,*,#55626,.T.);
#77824=ORIENTED_EDGE('',*,*,#55627,.T.);
#77825=ORIENTED_EDGE('',*,*,#55628,.T.);
#77826=ORIENTED_EDGE('',*,*,#55629,.T.);
#77827=ORIENTED_EDGE('',*,*,#55630,.T.);
#77828=ORIENTED_EDGE('',*,*,#55631,.T.);
#77829=ORIENTED_EDGE('',*,*,#55632,.T.);
#77830=ORIENTED_EDGE('',*,*,#55633,.T.);
#77831=ORIENTED_EDGE('',*,*,#55634,.T.);
#77832=ORIENTED_EDGE('',*,*,#55635,.T.);
#77833=ORIENTED_EDGE('',*,*,#55636,.T.);
#77834=ORIENTED_EDGE('',*,*,#55637,.T.);
#77835=ORIENTED_EDGE('',*,*,#55638,.T.);
#77836=ORIENTED_EDGE('',*,*,#55639,.T.);
#77837=ORIENTED_EDGE('',*,*,#55640,.T.);
#77838=ORIENTED_EDGE('',*,*,#55641,.T.);
#77839=ORIENTED_EDGE('',*,*,#55642,.T.);
#77840=ORIENTED_EDGE('',*,*,#55643,.T.);
#77841=ORIENTED_EDGE('',*,*,#55644,.T.);
#77842=ORIENTED_EDGE('',*,*,#55645,.T.);
#77843=ORIENTED_EDGE('',*,*,#55646,.T.);
#77844=ORIENTED_EDGE('',*,*,#55647,.T.);
#77845=ORIENTED_EDGE('',*,*,#55648,.T.);
#77846=ORIENTED_EDGE('',*,*,#55649,.T.);
#77847=ORIENTED_EDGE('',*,*,#55650,.T.);
#77848=ORIENTED_EDGE('',*,*,#55651,.T.);
#77849=ORIENTED_EDGE('',*,*,#55652,.T.);
#77850=ORIENTED_EDGE('',*,*,#55653,.T.);
#77851=ORIENTED_EDGE('',*,*,#55654,.T.);
#77852=ORIENTED_EDGE('',*,*,#55655,.T.);
#77853=ORIENTED_EDGE('',*,*,#55656,.T.);
#77854=ORIENTED_EDGE('',*,*,#55657,.T.);
#77855=ORIENTED_EDGE('',*,*,#55658,.T.);
#77856=ORIENTED_EDGE('',*,*,#55659,.T.);
#77857=ORIENTED_EDGE('',*,*,#55660,.T.);
#77858=ORIENTED_EDGE('',*,*,#55661,.T.);
#77859=ORIENTED_EDGE('',*,*,#55662,.T.);
#77860=ORIENTED_EDGE('',*,*,#55663,.T.);
#77861=ORIENTED_EDGE('',*,*,#55664,.T.);
#77862=ORIENTED_EDGE('',*,*,#55665,.T.);
#77863=ORIENTED_EDGE('',*,*,#55666,.T.);
#77864=ORIENTED_EDGE('',*,*,#55667,.T.);
#77865=ORIENTED_EDGE('',*,*,#55668,.T.);
#77866=ORIENTED_EDGE('',*,*,#55669,.T.);
#77867=ORIENTED_EDGE('',*,*,#55670,.T.);
#77868=ORIENTED_EDGE('',*,*,#55671,.T.);
#77869=ORIENTED_EDGE('',*,*,#55672,.T.);
#77870=ORIENTED_EDGE('',*,*,#55673,.T.);
#77871=ORIENTED_EDGE('',*,*,#55674,.T.);
#77872=ORIENTED_EDGE('',*,*,#55675,.T.);
#77873=ORIENTED_EDGE('',*,*,#55676,.T.);
#77874=ORIENTED_EDGE('',*,*,#55677,.T.);
#77875=ORIENTED_EDGE('',*,*,#55678,.T.);
#77876=ORIENTED_EDGE('',*,*,#55679,.T.);
#77877=ORIENTED_EDGE('',*,*,#55680,.T.);
#77878=ORIENTED_EDGE('',*,*,#55681,.T.);
#77879=ORIENTED_EDGE('',*,*,#55682,.T.);
#77880=ORIENTED_EDGE('',*,*,#55683,.T.);
#77881=ORIENTED_EDGE('',*,*,#55684,.T.);
#77882=ORIENTED_EDGE('',*,*,#55685,.T.);
#77883=ORIENTED_EDGE('',*,*,#55686,.T.);
#77884=ORIENTED_EDGE('',*,*,#55687,.T.);
#77885=ORIENTED_EDGE('',*,*,#55688,.T.);
#77886=ORIENTED_EDGE('',*,*,#55689,.T.);
#77887=ORIENTED_EDGE('',*,*,#55690,.T.);
#77888=ORIENTED_EDGE('',*,*,#55691,.T.);
#77889=ORIENTED_EDGE('',*,*,#55692,.T.);
#77890=ORIENTED_EDGE('',*,*,#55693,.T.);
#77891=ORIENTED_EDGE('',*,*,#55694,.T.);
#77892=ORIENTED_EDGE('',*,*,#55695,.T.);
#77893=ORIENTED_EDGE('',*,*,#55696,.T.);
#77894=ORIENTED_EDGE('',*,*,#55697,.T.);
#77895=ORIENTED_EDGE('',*,*,#55698,.T.);
#77896=ORIENTED_EDGE('',*,*,#55699,.T.);
#77897=ORIENTED_EDGE('',*,*,#55700,.T.);
#77898=ORIENTED_EDGE('',*,*,#55701,.T.);
#77899=ORIENTED_EDGE('',*,*,#55702,.T.);
#77900=ORIENTED_EDGE('',*,*,#55703,.T.);
#77901=ORIENTED_EDGE('',*,*,#55704,.T.);
#77902=ORIENTED_EDGE('',*,*,#55705,.T.);
#77903=ORIENTED_EDGE('',*,*,#55706,.T.);
#77904=ORIENTED_EDGE('',*,*,#55707,.T.);
#77905=ORIENTED_EDGE('',*,*,#55708,.T.);
#77906=ORIENTED_EDGE('',*,*,#55709,.T.);
#77907=ORIENTED_EDGE('',*,*,#55710,.T.);
#77908=ORIENTED_EDGE('',*,*,#55711,.T.);
#77909=ORIENTED_EDGE('',*,*,#55712,.T.);
#77910=ORIENTED_EDGE('',*,*,#55713,.T.);
#77911=ORIENTED_EDGE('',*,*,#55714,.T.);
#77912=ORIENTED_EDGE('',*,*,#55715,.T.);
#77913=ORIENTED_EDGE('',*,*,#55716,.T.);
#77914=ORIENTED_EDGE('',*,*,#55717,.T.);
#77915=ORIENTED_EDGE('',*,*,#55718,.T.);
#77916=ORIENTED_EDGE('',*,*,#55719,.T.);
#77917=ORIENTED_EDGE('',*,*,#55720,.T.);
#77918=ORIENTED_EDGE('',*,*,#55721,.T.);
#77919=ORIENTED_EDGE('',*,*,#55722,.T.);
#77920=ORIENTED_EDGE('',*,*,#55723,.T.);
#77921=ORIENTED_EDGE('',*,*,#55724,.T.);
#77922=ORIENTED_EDGE('',*,*,#55725,.T.);
#77923=ORIENTED_EDGE('',*,*,#55726,.T.);
#77924=ORIENTED_EDGE('',*,*,#55727,.T.);
#77925=ORIENTED_EDGE('',*,*,#55728,.T.);
#77926=ORIENTED_EDGE('',*,*,#55729,.T.);
#77927=ORIENTED_EDGE('',*,*,#55730,.T.);
#77928=ORIENTED_EDGE('',*,*,#55731,.T.);
#77929=ORIENTED_EDGE('',*,*,#55732,.T.);
#77930=ORIENTED_EDGE('',*,*,#55733,.T.);
#77931=ORIENTED_EDGE('',*,*,#55734,.T.);
#77932=ORIENTED_EDGE('',*,*,#55735,.T.);
#77933=ORIENTED_EDGE('',*,*,#55736,.T.);
#77934=ORIENTED_EDGE('',*,*,#55737,.T.);
#77935=ORIENTED_EDGE('',*,*,#55738,.T.);
#77936=ORIENTED_EDGE('',*,*,#55739,.T.);
#77937=ORIENTED_EDGE('',*,*,#55740,.T.);
#77938=ORIENTED_EDGE('',*,*,#55741,.T.);
#77939=ORIENTED_EDGE('',*,*,#55742,.T.);
#77940=ORIENTED_EDGE('',*,*,#55743,.T.);
#77941=ORIENTED_EDGE('',*,*,#55744,.T.);
#77942=ORIENTED_EDGE('',*,*,#55745,.T.);
#77943=ORIENTED_EDGE('',*,*,#55746,.T.);
#77944=ORIENTED_EDGE('',*,*,#55747,.T.);
#77945=ORIENTED_EDGE('',*,*,#55748,.T.);
#77946=ORIENTED_EDGE('',*,*,#55749,.T.);
#77947=ORIENTED_EDGE('',*,*,#55750,.T.);
#77948=ORIENTED_EDGE('',*,*,#55751,.T.);
#77949=ORIENTED_EDGE('',*,*,#55752,.T.);
#77950=ORIENTED_EDGE('',*,*,#55753,.T.);
#77951=ORIENTED_EDGE('',*,*,#55754,.T.);
#77952=ORIENTED_EDGE('',*,*,#55755,.T.);
#77953=ORIENTED_EDGE('',*,*,#55756,.T.);
#77954=ORIENTED_EDGE('',*,*,#55757,.T.);
#77955=ORIENTED_EDGE('',*,*,#55758,.T.);
#77956=ORIENTED_EDGE('',*,*,#55759,.T.);
#77957=ORIENTED_EDGE('',*,*,#55760,.T.);
#77958=ORIENTED_EDGE('',*,*,#55761,.T.);
#77959=ORIENTED_EDGE('',*,*,#55762,.T.);
#77960=ORIENTED_EDGE('',*,*,#55763,.T.);
#77961=ORIENTED_EDGE('',*,*,#55764,.T.);
#77962=ORIENTED_EDGE('',*,*,#55765,.T.);
#77963=ORIENTED_EDGE('',*,*,#55766,.T.);
#77964=ORIENTED_EDGE('',*,*,#55767,.T.);
#77965=ORIENTED_EDGE('',*,*,#55768,.T.);
#77966=ORIENTED_EDGE('',*,*,#55769,.T.);
#77967=ORIENTED_EDGE('',*,*,#55770,.T.);
#77968=ORIENTED_EDGE('',*,*,#55771,.T.);
#77969=ORIENTED_EDGE('',*,*,#55772,.T.);
#77970=ORIENTED_EDGE('',*,*,#55773,.T.);
#77971=ORIENTED_EDGE('',*,*,#55774,.T.);
#77972=ORIENTED_EDGE('',*,*,#55775,.T.);
#77973=ORIENTED_EDGE('',*,*,#55776,.T.);
#77974=ORIENTED_EDGE('',*,*,#55777,.T.);
#77975=ORIENTED_EDGE('',*,*,#55778,.T.);
#77976=ORIENTED_EDGE('',*,*,#55779,.T.);
#77977=ORIENTED_EDGE('',*,*,#55780,.T.);
#77978=ORIENTED_EDGE('',*,*,#55781,.T.);
#77979=ORIENTED_EDGE('',*,*,#55782,.T.);
#77980=ORIENTED_EDGE('',*,*,#55783,.T.);
#77981=ORIENTED_EDGE('',*,*,#55784,.T.);
#77982=ORIENTED_EDGE('',*,*,#55785,.T.);
#77983=ORIENTED_EDGE('',*,*,#55786,.T.);
#77984=ORIENTED_EDGE('',*,*,#55787,.T.);
#77985=ORIENTED_EDGE('',*,*,#55788,.T.);
#77986=ORIENTED_EDGE('',*,*,#55789,.T.);
#77987=ORIENTED_EDGE('',*,*,#55790,.T.);
#77988=ORIENTED_EDGE('',*,*,#55791,.T.);
#77989=ORIENTED_EDGE('',*,*,#55792,.T.);
#77990=ORIENTED_EDGE('',*,*,#55793,.T.);
#77991=ORIENTED_EDGE('',*,*,#55794,.T.);
#77992=ORIENTED_EDGE('',*,*,#55795,.T.);
#77993=ORIENTED_EDGE('',*,*,#55796,.T.);
#77994=ORIENTED_EDGE('',*,*,#55797,.T.);
#77995=ORIENTED_EDGE('',*,*,#55798,.T.);
#77996=ORIENTED_EDGE('',*,*,#55799,.T.);
#77997=ORIENTED_EDGE('',*,*,#55800,.T.);
#77998=ORIENTED_EDGE('',*,*,#55801,.T.);
#77999=ORIENTED_EDGE('',*,*,#55802,.T.);
#78000=ORIENTED_EDGE('',*,*,#55803,.T.);
#78001=ORIENTED_EDGE('',*,*,#55804,.T.);
#78002=ORIENTED_EDGE('',*,*,#55805,.T.);
#78003=ORIENTED_EDGE('',*,*,#55806,.T.);
#78004=ORIENTED_EDGE('',*,*,#55807,.T.);
#78005=ORIENTED_EDGE('',*,*,#55808,.T.);
#78006=ORIENTED_EDGE('',*,*,#55809,.T.);
#78007=ORIENTED_EDGE('',*,*,#55810,.T.);
#78008=ORIENTED_EDGE('',*,*,#55811,.T.);
#78009=ORIENTED_EDGE('',*,*,#55812,.T.);
#78010=ORIENTED_EDGE('',*,*,#55813,.T.);
#78011=ORIENTED_EDGE('',*,*,#55814,.T.);
#78012=ORIENTED_EDGE('',*,*,#55815,.T.);
#78013=ORIENTED_EDGE('',*,*,#55816,.T.);
#78014=ORIENTED_EDGE('',*,*,#55817,.T.);
#78015=ORIENTED_EDGE('',*,*,#55818,.T.);
#78016=ORIENTED_EDGE('',*,*,#55819,.T.);
#78017=ORIENTED_EDGE('',*,*,#55820,.T.);
#78018=ORIENTED_EDGE('',*,*,#55821,.T.);
#78019=ORIENTED_EDGE('',*,*,#55822,.T.);
#78020=ORIENTED_EDGE('',*,*,#55823,.T.);
#78021=ORIENTED_EDGE('',*,*,#55824,.T.);
#78022=ORIENTED_EDGE('',*,*,#55825,.T.);
#78023=ORIENTED_EDGE('',*,*,#55826,.T.);
#78024=ORIENTED_EDGE('',*,*,#55827,.T.);
#78025=ORIENTED_EDGE('',*,*,#55828,.T.);
#78026=ORIENTED_EDGE('',*,*,#55829,.T.);
#78027=ORIENTED_EDGE('',*,*,#55830,.T.);
#78028=ORIENTED_EDGE('',*,*,#55831,.T.);
#78029=ORIENTED_EDGE('',*,*,#55832,.T.);
#78030=ORIENTED_EDGE('',*,*,#55833,.T.);
#78031=ORIENTED_EDGE('',*,*,#55834,.T.);
#78032=ORIENTED_EDGE('',*,*,#55835,.T.);
#78033=ORIENTED_EDGE('',*,*,#55836,.T.);
#78034=ORIENTED_EDGE('',*,*,#55837,.T.);
#78035=ORIENTED_EDGE('',*,*,#55838,.T.);
#78036=ORIENTED_EDGE('',*,*,#55839,.T.);
#78037=ORIENTED_EDGE('',*,*,#55840,.T.);
#78038=ORIENTED_EDGE('',*,*,#55841,.T.);
#78039=ORIENTED_EDGE('',*,*,#55842,.T.);
#78040=ORIENTED_EDGE('',*,*,#55843,.T.);
#78041=ORIENTED_EDGE('',*,*,#55844,.T.);
#78042=ORIENTED_EDGE('',*,*,#55845,.T.);
#78043=ORIENTED_EDGE('',*,*,#55846,.T.);
#78044=ORIENTED_EDGE('',*,*,#55847,.T.);
#78045=ORIENTED_EDGE('',*,*,#55848,.T.);
#78046=ORIENTED_EDGE('',*,*,#55849,.T.);
#78047=ORIENTED_EDGE('',*,*,#55850,.T.);
#78048=ORIENTED_EDGE('',*,*,#55851,.T.);
#78049=ORIENTED_EDGE('',*,*,#55852,.T.);
#78050=ORIENTED_EDGE('',*,*,#55853,.T.);
#78051=ORIENTED_EDGE('',*,*,#55854,.T.);
#78052=ORIENTED_EDGE('',*,*,#55855,.T.);
#78053=ORIENTED_EDGE('',*,*,#55856,.T.);
#78054=ORIENTED_EDGE('',*,*,#55857,.T.);
#78055=ORIENTED_EDGE('',*,*,#55858,.T.);
#78056=ORIENTED_EDGE('',*,*,#55859,.T.);
#78057=ORIENTED_EDGE('',*,*,#55860,.T.);
#78058=ORIENTED_EDGE('',*,*,#55861,.T.);
#78059=ORIENTED_EDGE('',*,*,#55862,.T.);
#78060=ORIENTED_EDGE('',*,*,#55863,.T.);
#78061=ORIENTED_EDGE('',*,*,#55864,.T.);
#78062=ORIENTED_EDGE('',*,*,#55865,.T.);
#78063=ORIENTED_EDGE('',*,*,#55866,.T.);
#78064=ORIENTED_EDGE('',*,*,#55867,.T.);
#78065=ORIENTED_EDGE('',*,*,#55868,.T.);
#78066=ORIENTED_EDGE('',*,*,#55869,.T.);
#78067=ORIENTED_EDGE('',*,*,#55870,.T.);
#78068=ORIENTED_EDGE('',*,*,#55871,.T.);
#78069=ORIENTED_EDGE('',*,*,#55872,.T.);
#78070=ORIENTED_EDGE('',*,*,#55873,.T.);
#78071=ORIENTED_EDGE('',*,*,#55874,.T.);
#78072=ORIENTED_EDGE('',*,*,#55875,.T.);
#78073=ORIENTED_EDGE('',*,*,#55876,.T.);
#78074=ORIENTED_EDGE('',*,*,#55877,.T.);
#78075=ORIENTED_EDGE('',*,*,#55878,.T.);
#78076=ORIENTED_EDGE('',*,*,#52035,.T.);
#78077=ORIENTED_EDGE('',*,*,#55879,.T.);
#78078=ORIENTED_EDGE('',*,*,#52029,.T.);
#78079=ORIENTED_EDGE('',*,*,#55880,.T.);
#78080=ORIENTED_EDGE('',*,*,#55881,.T.);
#78081=ORIENTED_EDGE('',*,*,#55882,.T.);
#78082=ORIENTED_EDGE('',*,*,#55883,.T.);
#78083=ORIENTED_EDGE('',*,*,#55884,.T.);
#78084=ORIENTED_EDGE('',*,*,#55885,.T.);
#78085=ORIENTED_EDGE('',*,*,#55886,.T.);
#78086=ORIENTED_EDGE('',*,*,#55887,.T.);
#78087=ORIENTED_EDGE('',*,*,#55888,.T.);
#78088=ORIENTED_EDGE('',*,*,#55889,.T.);
#78089=ORIENTED_EDGE('',*,*,#55890,.T.);
#78090=ORIENTED_EDGE('',*,*,#55891,.T.);
#78091=ORIENTED_EDGE('',*,*,#55892,.T.);
#78092=ORIENTED_EDGE('',*,*,#55893,.T.);
#78093=ORIENTED_EDGE('',*,*,#55894,.T.);
#78094=ORIENTED_EDGE('',*,*,#55895,.T.);
#78095=ORIENTED_EDGE('',*,*,#55896,.T.);
#78096=ORIENTED_EDGE('',*,*,#55897,.T.);
#78097=ORIENTED_EDGE('',*,*,#55898,.T.);
#78098=ORIENTED_EDGE('',*,*,#55899,.T.);
#78099=ORIENTED_EDGE('',*,*,#55900,.T.);
#78100=ORIENTED_EDGE('',*,*,#55901,.T.);
#78101=ORIENTED_EDGE('',*,*,#55902,.T.);
#78102=ORIENTED_EDGE('',*,*,#55903,.T.);
#78103=ORIENTED_EDGE('',*,*,#55904,.T.);
#78104=ORIENTED_EDGE('',*,*,#55905,.T.);
#78105=ORIENTED_EDGE('',*,*,#55906,.T.);
#78106=ORIENTED_EDGE('',*,*,#55907,.T.);
#78107=ORIENTED_EDGE('',*,*,#55908,.T.);
#78108=ORIENTED_EDGE('',*,*,#55909,.T.);
#78109=ORIENTED_EDGE('',*,*,#55910,.T.);
#78110=ORIENTED_EDGE('',*,*,#55911,.T.);
#78111=ORIENTED_EDGE('',*,*,#55912,.T.);
#78112=ORIENTED_EDGE('',*,*,#55913,.T.);
#78113=ORIENTED_EDGE('',*,*,#55914,.T.);
#78114=ORIENTED_EDGE('',*,*,#55915,.T.);
#78115=ORIENTED_EDGE('',*,*,#55916,.T.);
#78116=ORIENTED_EDGE('',*,*,#55917,.T.);
#78117=ORIENTED_EDGE('',*,*,#55918,.T.);
#78118=ORIENTED_EDGE('',*,*,#55919,.T.);
#78119=ORIENTED_EDGE('',*,*,#55920,.T.);
#78120=ORIENTED_EDGE('',*,*,#55921,.T.);
#78121=ORIENTED_EDGE('',*,*,#55922,.T.);
#78122=ORIENTED_EDGE('',*,*,#55923,.T.);
#78123=ORIENTED_EDGE('',*,*,#55924,.T.);
#78124=ORIENTED_EDGE('',*,*,#55925,.T.);
#78125=ORIENTED_EDGE('',*,*,#55926,.T.);
#78126=ORIENTED_EDGE('',*,*,#55927,.T.);
#78127=ORIENTED_EDGE('',*,*,#55928,.T.);
#78128=ORIENTED_EDGE('',*,*,#55929,.T.);
#78129=ORIENTED_EDGE('',*,*,#55930,.T.);
#78130=ORIENTED_EDGE('',*,*,#55931,.T.);
#78131=ORIENTED_EDGE('',*,*,#55932,.T.);
#78132=ORIENTED_EDGE('',*,*,#55933,.T.);
#78133=ORIENTED_EDGE('',*,*,#55934,.T.);
#78134=ORIENTED_EDGE('',*,*,#55935,.T.);
#78135=ORIENTED_EDGE('',*,*,#55936,.T.);
#78136=ORIENTED_EDGE('',*,*,#55937,.T.);
#78137=ORIENTED_EDGE('',*,*,#55938,.T.);
#78138=ORIENTED_EDGE('',*,*,#55939,.T.);
#78139=ORIENTED_EDGE('',*,*,#55940,.T.);
#78140=ORIENTED_EDGE('',*,*,#55941,.T.);
#78141=ORIENTED_EDGE('',*,*,#55942,.T.);
#78142=ORIENTED_EDGE('',*,*,#55943,.T.);
#78143=ORIENTED_EDGE('',*,*,#55944,.T.);
#78144=ORIENTED_EDGE('',*,*,#55945,.T.);
#78145=ORIENTED_EDGE('',*,*,#55946,.T.);
#78146=ORIENTED_EDGE('',*,*,#55947,.T.);
#78147=ORIENTED_EDGE('',*,*,#55948,.T.);
#78148=ORIENTED_EDGE('',*,*,#55949,.T.);
#78149=ORIENTED_EDGE('',*,*,#55950,.T.);
#78150=ORIENTED_EDGE('',*,*,#55951,.T.);
#78151=ORIENTED_EDGE('',*,*,#55952,.T.);
#78152=ORIENTED_EDGE('',*,*,#55953,.T.);
#78153=ORIENTED_EDGE('',*,*,#55954,.T.);
#78154=ORIENTED_EDGE('',*,*,#55955,.T.);
#78155=ORIENTED_EDGE('',*,*,#55956,.T.);
#78156=ORIENTED_EDGE('',*,*,#55957,.T.);
#78157=ORIENTED_EDGE('',*,*,#55958,.T.);
#78158=ORIENTED_EDGE('',*,*,#55959,.T.);
#78159=ORIENTED_EDGE('',*,*,#55960,.T.);
#78160=ORIENTED_EDGE('',*,*,#55961,.T.);
#78161=ORIENTED_EDGE('',*,*,#55962,.T.);
#78162=ORIENTED_EDGE('',*,*,#55963,.T.);
#78163=ORIENTED_EDGE('',*,*,#55964,.T.);
#78164=ORIENTED_EDGE('',*,*,#55965,.T.);
#78165=ORIENTED_EDGE('',*,*,#55966,.T.);
#78166=ORIENTED_EDGE('',*,*,#55967,.T.);
#78167=ORIENTED_EDGE('',*,*,#55968,.T.);
#78168=ORIENTED_EDGE('',*,*,#55969,.T.);
#78169=ORIENTED_EDGE('',*,*,#55970,.T.);
#78170=ORIENTED_EDGE('',*,*,#55971,.T.);
#78171=ORIENTED_EDGE('',*,*,#55972,.T.);
#78172=ORIENTED_EDGE('',*,*,#55973,.T.);
#78173=ORIENTED_EDGE('',*,*,#55974,.T.);
#78174=ORIENTED_EDGE('',*,*,#55975,.T.);
#78175=ORIENTED_EDGE('',*,*,#55976,.T.);
#78176=ORIENTED_EDGE('',*,*,#55977,.T.);
#78177=ORIENTED_EDGE('',*,*,#55978,.T.);
#78178=ORIENTED_EDGE('',*,*,#55979,.T.);
#78179=ORIENTED_EDGE('',*,*,#55980,.T.);
#78180=ORIENTED_EDGE('',*,*,#55981,.T.);
#78181=ORIENTED_EDGE('',*,*,#55982,.T.);
#78182=ORIENTED_EDGE('',*,*,#55983,.T.);
#78183=ORIENTED_EDGE('',*,*,#55984,.T.);
#78184=ORIENTED_EDGE('',*,*,#55985,.T.);
#78185=ORIENTED_EDGE('',*,*,#55986,.T.);
#78186=ORIENTED_EDGE('',*,*,#55987,.T.);
#78187=ORIENTED_EDGE('',*,*,#55988,.T.);
#78188=ORIENTED_EDGE('',*,*,#55989,.T.);
#78189=ORIENTED_EDGE('',*,*,#55990,.T.);
#78190=ORIENTED_EDGE('',*,*,#55991,.T.);
#78191=ORIENTED_EDGE('',*,*,#55992,.T.);
#78192=ORIENTED_EDGE('',*,*,#55993,.T.);
#78193=ORIENTED_EDGE('',*,*,#55994,.T.);
#78194=ORIENTED_EDGE('',*,*,#55995,.T.);
#78195=ORIENTED_EDGE('',*,*,#55996,.T.);
#78196=ORIENTED_EDGE('',*,*,#55997,.T.);
#78197=ORIENTED_EDGE('',*,*,#55998,.T.);
#78198=ORIENTED_EDGE('',*,*,#55999,.T.);
#78199=ORIENTED_EDGE('',*,*,#56000,.T.);
#78200=ORIENTED_EDGE('',*,*,#56001,.T.);
#78201=ORIENTED_EDGE('',*,*,#56002,.T.);
#78202=ORIENTED_EDGE('',*,*,#56003,.T.);
#78203=ORIENTED_EDGE('',*,*,#56004,.T.);
#78204=ORIENTED_EDGE('',*,*,#56005,.T.);
#78205=ORIENTED_EDGE('',*,*,#56006,.T.);
#78206=ORIENTED_EDGE('',*,*,#56007,.T.);
#78207=ORIENTED_EDGE('',*,*,#56008,.T.);
#78208=ORIENTED_EDGE('',*,*,#56009,.T.);
#78209=ORIENTED_EDGE('',*,*,#56010,.T.);
#78210=ORIENTED_EDGE('',*,*,#56011,.T.);
#78211=ORIENTED_EDGE('',*,*,#56012,.T.);
#78212=ORIENTED_EDGE('',*,*,#56013,.T.);
#78213=ORIENTED_EDGE('',*,*,#56014,.T.);
#78214=ORIENTED_EDGE('',*,*,#56015,.T.);
#78215=ORIENTED_EDGE('',*,*,#56016,.T.);
#78216=ORIENTED_EDGE('',*,*,#56017,.T.);
#78217=ORIENTED_EDGE('',*,*,#56018,.T.);
#78218=ORIENTED_EDGE('',*,*,#56019,.T.);
#78219=ORIENTED_EDGE('',*,*,#56020,.T.);
#78220=ORIENTED_EDGE('',*,*,#56021,.T.);
#78221=ORIENTED_EDGE('',*,*,#56022,.T.);
#78222=ORIENTED_EDGE('',*,*,#56023,.T.);
#78223=ORIENTED_EDGE('',*,*,#56024,.T.);
#78224=ORIENTED_EDGE('',*,*,#56025,.T.);
#78225=ORIENTED_EDGE('',*,*,#56026,.T.);
#78226=ORIENTED_EDGE('',*,*,#56027,.T.);
#78227=ORIENTED_EDGE('',*,*,#56028,.T.);
#78228=ORIENTED_EDGE('',*,*,#56029,.T.);
#78229=ORIENTED_EDGE('',*,*,#56030,.T.);
#78230=ORIENTED_EDGE('',*,*,#56031,.T.);
#78231=ORIENTED_EDGE('',*,*,#56032,.T.);
#78232=ORIENTED_EDGE('',*,*,#56033,.T.);
#78233=ORIENTED_EDGE('',*,*,#56034,.T.);
#78234=ORIENTED_EDGE('',*,*,#56035,.T.);
#78235=ORIENTED_EDGE('',*,*,#56036,.T.);
#78236=ORIENTED_EDGE('',*,*,#56037,.T.);
#78237=ORIENTED_EDGE('',*,*,#56038,.T.);
#78238=ORIENTED_EDGE('',*,*,#56039,.T.);
#78239=ORIENTED_EDGE('',*,*,#56040,.T.);
#78240=ORIENTED_EDGE('',*,*,#56041,.T.);
#78241=ORIENTED_EDGE('',*,*,#56042,.T.);
#78242=ORIENTED_EDGE('',*,*,#56043,.T.);
#78243=ORIENTED_EDGE('',*,*,#56044,.T.);
#78244=ORIENTED_EDGE('',*,*,#56045,.T.);
#78245=ORIENTED_EDGE('',*,*,#56046,.T.);
#78246=ORIENTED_EDGE('',*,*,#56047,.T.);
#78247=ORIENTED_EDGE('',*,*,#56048,.T.);
#78248=ORIENTED_EDGE('',*,*,#56049,.T.);
#78249=ORIENTED_EDGE('',*,*,#56050,.T.);
#78250=ORIENTED_EDGE('',*,*,#56051,.T.);
#78251=ORIENTED_EDGE('',*,*,#56052,.T.);
#78252=ORIENTED_EDGE('',*,*,#56053,.T.);
#78253=ORIENTED_EDGE('',*,*,#56054,.T.);
#78254=ORIENTED_EDGE('',*,*,#56055,.T.);
#78255=ORIENTED_EDGE('',*,*,#56056,.T.);
#78256=ORIENTED_EDGE('',*,*,#56057,.T.);
#78257=ORIENTED_EDGE('',*,*,#56058,.T.);
#78258=ORIENTED_EDGE('',*,*,#56059,.T.);
#78259=ORIENTED_EDGE('',*,*,#56060,.T.);
#78260=ORIENTED_EDGE('',*,*,#56061,.T.);
#78261=ORIENTED_EDGE('',*,*,#56062,.T.);
#78262=ORIENTED_EDGE('',*,*,#56063,.T.);
#78263=ORIENTED_EDGE('',*,*,#56064,.T.);
#78264=ORIENTED_EDGE('',*,*,#56065,.T.);
#78265=ORIENTED_EDGE('',*,*,#56066,.T.);
#78266=ORIENTED_EDGE('',*,*,#56067,.T.);
#78267=ORIENTED_EDGE('',*,*,#56068,.T.);
#78268=ORIENTED_EDGE('',*,*,#56069,.T.);
#78269=ORIENTED_EDGE('',*,*,#56070,.T.);
#78270=ORIENTED_EDGE('',*,*,#56071,.T.);
#78271=ORIENTED_EDGE('',*,*,#56072,.T.);
#78272=ORIENTED_EDGE('',*,*,#56073,.T.);
#78273=ORIENTED_EDGE('',*,*,#56074,.T.);
#78274=ORIENTED_EDGE('',*,*,#56075,.T.);
#78275=ORIENTED_EDGE('',*,*,#56076,.T.);
#78276=ORIENTED_EDGE('',*,*,#56077,.T.);
#78277=ORIENTED_EDGE('',*,*,#56078,.T.);
#78278=ORIENTED_EDGE('',*,*,#56079,.T.);
#78279=ORIENTED_EDGE('',*,*,#56080,.T.);
#78280=ORIENTED_EDGE('',*,*,#56081,.T.);
#78281=ORIENTED_EDGE('',*,*,#56082,.T.);
#78282=ORIENTED_EDGE('',*,*,#56083,.T.);
#78283=ORIENTED_EDGE('',*,*,#56084,.T.);
#78284=ORIENTED_EDGE('',*,*,#56085,.T.);
#78285=ORIENTED_EDGE('',*,*,#56086,.T.);
#78286=ORIENTED_EDGE('',*,*,#56087,.T.);
#78287=ORIENTED_EDGE('',*,*,#56088,.T.);
#78288=ORIENTED_EDGE('',*,*,#56089,.T.);
#78289=ORIENTED_EDGE('',*,*,#56090,.T.);
#78290=ORIENTED_EDGE('',*,*,#56091,.T.);
#78291=ORIENTED_EDGE('',*,*,#56092,.T.);
#78292=ORIENTED_EDGE('',*,*,#56093,.T.);
#78293=ORIENTED_EDGE('',*,*,#56094,.T.);
#78294=ORIENTED_EDGE('',*,*,#56095,.T.);
#78295=ORIENTED_EDGE('',*,*,#56096,.T.);
#78296=ORIENTED_EDGE('',*,*,#56097,.T.);
#78297=ORIENTED_EDGE('',*,*,#56098,.T.);
#78298=ORIENTED_EDGE('',*,*,#56099,.T.);
#78299=ORIENTED_EDGE('',*,*,#56100,.T.);
#78300=ORIENTED_EDGE('',*,*,#56101,.T.);
#78301=ORIENTED_EDGE('',*,*,#56102,.T.);
#78302=ORIENTED_EDGE('',*,*,#56103,.T.);
#78303=ORIENTED_EDGE('',*,*,#56104,.T.);
#78304=ORIENTED_EDGE('',*,*,#56105,.T.);
#78305=ORIENTED_EDGE('',*,*,#56106,.T.);
#78306=ORIENTED_EDGE('',*,*,#56107,.T.);
#78307=ORIENTED_EDGE('',*,*,#56108,.T.);
#78308=ORIENTED_EDGE('',*,*,#56109,.T.);
#78309=ORIENTED_EDGE('',*,*,#56110,.T.);
#78310=ORIENTED_EDGE('',*,*,#56111,.T.);
#78311=ORIENTED_EDGE('',*,*,#56112,.T.);
#78312=ORIENTED_EDGE('',*,*,#56113,.T.);
#78313=ORIENTED_EDGE('',*,*,#56114,.T.);
#78314=ORIENTED_EDGE('',*,*,#56115,.T.);
#78315=ORIENTED_EDGE('',*,*,#56116,.T.);
#78316=ORIENTED_EDGE('',*,*,#56117,.T.);
#78317=ORIENTED_EDGE('',*,*,#56118,.T.);
#78318=ORIENTED_EDGE('',*,*,#56119,.T.);
#78319=ORIENTED_EDGE('',*,*,#56120,.T.);
#78320=ORIENTED_EDGE('',*,*,#56121,.T.);
#78321=ORIENTED_EDGE('',*,*,#56122,.T.);
#78322=ORIENTED_EDGE('',*,*,#56123,.T.);
#78323=ORIENTED_EDGE('',*,*,#56124,.T.);
#78324=ORIENTED_EDGE('',*,*,#56125,.T.);
#78325=ORIENTED_EDGE('',*,*,#56126,.T.);
#78326=ORIENTED_EDGE('',*,*,#56127,.T.);
#78327=ORIENTED_EDGE('',*,*,#56128,.T.);
#78328=ORIENTED_EDGE('',*,*,#56129,.T.);
#78329=ORIENTED_EDGE('',*,*,#56130,.T.);
#78330=ORIENTED_EDGE('',*,*,#56131,.T.);
#78331=ORIENTED_EDGE('',*,*,#56132,.T.);
#78332=ORIENTED_EDGE('',*,*,#56133,.T.);
#78333=ORIENTED_EDGE('',*,*,#56134,.T.);
#78334=ORIENTED_EDGE('',*,*,#56135,.T.);
#78335=ORIENTED_EDGE('',*,*,#56136,.T.);
#78336=ORIENTED_EDGE('',*,*,#56137,.T.);
#78337=ORIENTED_EDGE('',*,*,#56138,.T.);
#78338=ORIENTED_EDGE('',*,*,#56139,.T.);
#78339=ORIENTED_EDGE('',*,*,#56140,.T.);
#78340=ORIENTED_EDGE('',*,*,#56141,.T.);
#78341=ORIENTED_EDGE('',*,*,#56142,.T.);
#78342=ORIENTED_EDGE('',*,*,#56143,.T.);
#78343=ORIENTED_EDGE('',*,*,#56144,.T.);
#78344=ORIENTED_EDGE('',*,*,#56145,.T.);
#78345=ORIENTED_EDGE('',*,*,#56146,.T.);
#78346=ORIENTED_EDGE('',*,*,#56147,.T.);
#78347=ORIENTED_EDGE('',*,*,#56148,.T.);
#78348=ORIENTED_EDGE('',*,*,#56149,.T.);
#78349=ORIENTED_EDGE('',*,*,#56150,.T.);
#78350=ORIENTED_EDGE('',*,*,#56151,.T.);
#78351=ORIENTED_EDGE('',*,*,#56152,.T.);
#78352=ORIENTED_EDGE('',*,*,#56153,.T.);
#78353=ORIENTED_EDGE('',*,*,#56154,.T.);
#78354=ORIENTED_EDGE('',*,*,#56155,.T.);
#78355=ORIENTED_EDGE('',*,*,#56156,.T.);
#78356=ORIENTED_EDGE('',*,*,#56157,.T.);
#78357=ORIENTED_EDGE('',*,*,#56158,.T.);
#78358=ORIENTED_EDGE('',*,*,#56159,.T.);
#78359=ORIENTED_EDGE('',*,*,#56160,.T.);
#78360=ORIENTED_EDGE('',*,*,#56161,.T.);
#78361=ORIENTED_EDGE('',*,*,#56162,.T.);
#78362=ORIENTED_EDGE('',*,*,#56163,.T.);
#78363=ORIENTED_EDGE('',*,*,#56164,.T.);
#78364=ORIENTED_EDGE('',*,*,#56165,.T.);
#78365=ORIENTED_EDGE('',*,*,#56166,.T.);
#78366=ORIENTED_EDGE('',*,*,#56167,.T.);
#78367=ORIENTED_EDGE('',*,*,#56168,.T.);
#78368=ORIENTED_EDGE('',*,*,#56169,.T.);
#78369=ORIENTED_EDGE('',*,*,#56170,.T.);
#78370=ORIENTED_EDGE('',*,*,#56171,.T.);
#78371=ORIENTED_EDGE('',*,*,#56172,.T.);
#78372=ORIENTED_EDGE('',*,*,#56173,.T.);
#78373=ORIENTED_EDGE('',*,*,#56174,.T.);
#78374=ORIENTED_EDGE('',*,*,#56175,.T.);
#78375=ORIENTED_EDGE('',*,*,#56176,.T.);
#78376=ORIENTED_EDGE('',*,*,#56177,.T.);
#78377=ORIENTED_EDGE('',*,*,#56178,.T.);
#78378=ORIENTED_EDGE('',*,*,#56179,.T.);
#78379=ORIENTED_EDGE('',*,*,#56180,.T.);
#78380=ORIENTED_EDGE('',*,*,#56181,.T.);
#78381=ORIENTED_EDGE('',*,*,#56182,.T.);
#78382=ORIENTED_EDGE('',*,*,#56183,.T.);
#78383=ORIENTED_EDGE('',*,*,#56184,.T.);
#78384=ORIENTED_EDGE('',*,*,#56185,.T.);
#78385=ORIENTED_EDGE('',*,*,#56186,.T.);
#78386=ORIENTED_EDGE('',*,*,#56187,.T.);
#78387=ORIENTED_EDGE('',*,*,#56188,.T.);
#78388=ORIENTED_EDGE('',*,*,#56189,.T.);
#78389=ORIENTED_EDGE('',*,*,#56190,.T.);
#78390=ORIENTED_EDGE('',*,*,#56191,.T.);
#78391=ORIENTED_EDGE('',*,*,#56192,.T.);
#78392=ORIENTED_EDGE('',*,*,#56193,.T.);
#78393=ORIENTED_EDGE('',*,*,#56194,.T.);
#78394=ORIENTED_EDGE('',*,*,#56195,.T.);
#78395=ORIENTED_EDGE('',*,*,#56196,.T.);
#78396=ORIENTED_EDGE('',*,*,#56197,.T.);
#78397=ORIENTED_EDGE('',*,*,#56198,.T.);
#78398=ORIENTED_EDGE('',*,*,#56199,.T.);
#78399=ORIENTED_EDGE('',*,*,#56200,.T.);
#78400=ORIENTED_EDGE('',*,*,#56201,.T.);
#78401=ORIENTED_EDGE('',*,*,#56202,.T.);
#78402=ORIENTED_EDGE('',*,*,#56203,.T.);
#78403=ORIENTED_EDGE('',*,*,#56204,.T.);
#78404=ORIENTED_EDGE('',*,*,#56205,.T.);
#78405=ORIENTED_EDGE('',*,*,#56206,.T.);
#78406=ORIENTED_EDGE('',*,*,#56207,.T.);
#78407=ORIENTED_EDGE('',*,*,#56208,.T.);
#78408=ORIENTED_EDGE('',*,*,#56209,.T.);
#78409=ORIENTED_EDGE('',*,*,#56210,.T.);
#78410=ORIENTED_EDGE('',*,*,#56211,.T.);
#78411=ORIENTED_EDGE('',*,*,#56212,.T.);
#78412=ORIENTED_EDGE('',*,*,#56213,.T.);
#78413=ORIENTED_EDGE('',*,*,#56214,.T.);
#78414=ORIENTED_EDGE('',*,*,#56215,.T.);
#78415=ORIENTED_EDGE('',*,*,#56216,.T.);
#78416=ORIENTED_EDGE('',*,*,#56217,.T.);
#78417=ORIENTED_EDGE('',*,*,#56218,.T.);
#78418=ORIENTED_EDGE('',*,*,#56219,.T.);
#78419=ORIENTED_EDGE('',*,*,#56220,.T.);
#78420=ORIENTED_EDGE('',*,*,#56221,.T.);
#78421=ORIENTED_EDGE('',*,*,#56222,.T.);
#78422=ORIENTED_EDGE('',*,*,#56223,.T.);
#78423=ORIENTED_EDGE('',*,*,#56224,.T.);
#78424=ORIENTED_EDGE('',*,*,#56225,.T.);
#78425=ORIENTED_EDGE('',*,*,#56226,.T.);
#78426=ORIENTED_EDGE('',*,*,#56227,.T.);
#78427=ORIENTED_EDGE('',*,*,#56228,.T.);
#78428=ORIENTED_EDGE('',*,*,#56229,.T.);
#78429=ORIENTED_EDGE('',*,*,#56230,.T.);
#78430=ORIENTED_EDGE('',*,*,#56231,.T.);
#78431=ORIENTED_EDGE('',*,*,#56232,.T.);
#78432=ORIENTED_EDGE('',*,*,#56233,.T.);
#78433=ORIENTED_EDGE('',*,*,#56234,.T.);
#78434=ORIENTED_EDGE('',*,*,#56235,.T.);
#78435=ORIENTED_EDGE('',*,*,#56236,.T.);
#78436=ORIENTED_EDGE('',*,*,#56237,.T.);
#78437=ORIENTED_EDGE('',*,*,#56238,.T.);
#78438=ORIENTED_EDGE('',*,*,#56239,.T.);
#78439=ORIENTED_EDGE('',*,*,#56240,.T.);
#78440=ORIENTED_EDGE('',*,*,#56241,.T.);
#78441=ORIENTED_EDGE('',*,*,#56242,.T.);
#78442=ORIENTED_EDGE('',*,*,#56243,.T.);
#78443=ORIENTED_EDGE('',*,*,#56244,.T.);
#78444=ORIENTED_EDGE('',*,*,#56245,.T.);
#78445=ORIENTED_EDGE('',*,*,#56246,.T.);
#78446=ORIENTED_EDGE('',*,*,#56247,.T.);
#78447=ORIENTED_EDGE('',*,*,#56248,.T.);
#78448=ORIENTED_EDGE('',*,*,#56249,.T.);
#78449=ORIENTED_EDGE('',*,*,#56250,.T.);
#78450=ORIENTED_EDGE('',*,*,#56251,.T.);
#78451=ORIENTED_EDGE('',*,*,#56252,.T.);
#78452=ORIENTED_EDGE('',*,*,#56253,.T.);
#78453=ORIENTED_EDGE('',*,*,#56254,.T.);
#78454=ORIENTED_EDGE('',*,*,#56255,.T.);
#78455=ORIENTED_EDGE('',*,*,#56256,.T.);
#78456=ORIENTED_EDGE('',*,*,#56257,.T.);
#78457=ORIENTED_EDGE('',*,*,#56258,.T.);
#78458=ORIENTED_EDGE('',*,*,#56259,.T.);
#78459=ORIENTED_EDGE('',*,*,#56260,.T.);
#78460=ORIENTED_EDGE('',*,*,#56261,.T.);
#78461=ORIENTED_EDGE('',*,*,#56262,.T.);
#78462=ORIENTED_EDGE('',*,*,#56263,.T.);
#78463=ORIENTED_EDGE('',*,*,#56264,.T.);
#78464=ORIENTED_EDGE('',*,*,#56265,.T.);
#78465=ORIENTED_EDGE('',*,*,#56266,.T.);
#78466=ORIENTED_EDGE('',*,*,#56267,.T.);
#78467=ORIENTED_EDGE('',*,*,#56268,.T.);
#78468=ORIENTED_EDGE('',*,*,#56269,.T.);
#78469=ORIENTED_EDGE('',*,*,#56270,.T.);
#78470=ORIENTED_EDGE('',*,*,#56271,.T.);
#78471=ORIENTED_EDGE('',*,*,#56272,.T.);
#78472=ORIENTED_EDGE('',*,*,#56273,.T.);
#78473=ORIENTED_EDGE('',*,*,#56274,.T.);
#78474=ORIENTED_EDGE('',*,*,#56275,.T.);
#78475=ORIENTED_EDGE('',*,*,#56276,.T.);
#78476=ORIENTED_EDGE('',*,*,#56277,.T.);
#78477=ORIENTED_EDGE('',*,*,#56278,.T.);
#78478=ORIENTED_EDGE('',*,*,#56279,.T.);
#78479=ORIENTED_EDGE('',*,*,#56280,.T.);
#78480=ORIENTED_EDGE('',*,*,#56281,.T.);
#78481=ORIENTED_EDGE('',*,*,#56282,.T.);
#78482=ORIENTED_EDGE('',*,*,#56283,.T.);
#78483=ORIENTED_EDGE('',*,*,#56284,.T.);
#78484=ORIENTED_EDGE('',*,*,#56285,.T.);
#78485=ORIENTED_EDGE('',*,*,#56286,.T.);
#78486=ORIENTED_EDGE('',*,*,#56287,.T.);
#78487=ORIENTED_EDGE('',*,*,#56288,.T.);
#78488=ORIENTED_EDGE('',*,*,#56289,.T.);
#78489=ORIENTED_EDGE('',*,*,#56290,.T.);
#78490=ORIENTED_EDGE('',*,*,#56291,.T.);
#78491=ORIENTED_EDGE('',*,*,#56292,.T.);
#78492=ORIENTED_EDGE('',*,*,#56293,.T.);
#78493=ORIENTED_EDGE('',*,*,#56294,.T.);
#78494=ORIENTED_EDGE('',*,*,#56295,.T.);
#78495=ORIENTED_EDGE('',*,*,#54666,.F.);
#78496=ORIENTED_EDGE('',*,*,#56296,.T.);
#78497=ORIENTED_EDGE('',*,*,#54648,.F.);
#78498=ORIENTED_EDGE('',*,*,#56297,.T.);
#78499=ORIENTED_EDGE('',*,*,#54650,.F.);
#78500=ORIENTED_EDGE('',*,*,#56298,.T.);
#78501=ORIENTED_EDGE('',*,*,#54654,.F.);
#78502=ORIENTED_EDGE('',*,*,#56299,.T.);
#78503=ORIENTED_EDGE('',*,*,#54694,.F.);
#78504=ORIENTED_EDGE('',*,*,#56300,.T.);
#78505=ORIENTED_EDGE('',*,*,#54676,.F.);
#78506=ORIENTED_EDGE('',*,*,#56301,.T.);
#78507=ORIENTED_EDGE('',*,*,#54678,.F.);
#78508=ORIENTED_EDGE('',*,*,#56302,.T.);
#78509=ORIENTED_EDGE('',*,*,#54682,.F.);
#78510=ORIENTED_EDGE('',*,*,#56303,.T.);
#78511=ORIENTED_EDGE('',*,*,#54722,.F.);
#78512=ORIENTED_EDGE('',*,*,#56304,.T.);
#78513=ORIENTED_EDGE('',*,*,#54704,.F.);
#78514=ORIENTED_EDGE('',*,*,#56305,.T.);
#78515=ORIENTED_EDGE('',*,*,#54706,.F.);
#78516=ORIENTED_EDGE('',*,*,#56306,.T.);
#78517=ORIENTED_EDGE('',*,*,#54710,.F.);
#78518=ORIENTED_EDGE('',*,*,#56307,.T.);
#78519=ORIENTED_EDGE('',*,*,#54750,.F.);
#78520=ORIENTED_EDGE('',*,*,#56308,.T.);
#78521=ORIENTED_EDGE('',*,*,#54732,.F.);
#78522=ORIENTED_EDGE('',*,*,#56309,.T.);
#78523=ORIENTED_EDGE('',*,*,#54734,.F.);
#78524=ORIENTED_EDGE('',*,*,#56310,.T.);
#78525=ORIENTED_EDGE('',*,*,#54738,.F.);
#78526=ORIENTED_EDGE('',*,*,#56311,.T.);
#78527=ORIENTED_EDGE('',*,*,#54778,.F.);
#78528=ORIENTED_EDGE('',*,*,#56312,.T.);
#78529=ORIENTED_EDGE('',*,*,#54760,.F.);
#78530=ORIENTED_EDGE('',*,*,#56313,.T.);
#78531=ORIENTED_EDGE('',*,*,#54762,.F.);
#78532=ORIENTED_EDGE('',*,*,#56314,.T.);
#78533=ORIENTED_EDGE('',*,*,#54766,.F.);
#78534=ORIENTED_EDGE('',*,*,#56315,.T.);
#78535=ORIENTED_EDGE('',*,*,#54806,.F.);
#78536=ORIENTED_EDGE('',*,*,#56316,.T.);
#78537=ORIENTED_EDGE('',*,*,#54788,.F.);
#78538=ORIENTED_EDGE('',*,*,#56317,.T.);
#78539=ORIENTED_EDGE('',*,*,#54790,.F.);
#78540=ORIENTED_EDGE('',*,*,#56318,.T.);
#78541=ORIENTED_EDGE('',*,*,#54794,.F.);
#78542=ORIENTED_EDGE('',*,*,#56319,.T.);
#78543=ORIENTED_EDGE('',*,*,#54834,.F.);
#78544=ORIENTED_EDGE('',*,*,#56320,.T.);
#78545=ORIENTED_EDGE('',*,*,#54816,.F.);
#78546=ORIENTED_EDGE('',*,*,#56321,.T.);
#78547=ORIENTED_EDGE('',*,*,#54818,.F.);
#78548=ORIENTED_EDGE('',*,*,#56322,.T.);
#78549=ORIENTED_EDGE('',*,*,#54822,.F.);
#78550=ORIENTED_EDGE('',*,*,#56323,.T.);
#78551=ORIENTED_EDGE('',*,*,#54862,.F.);
#78552=ORIENTED_EDGE('',*,*,#56324,.T.);
#78553=ORIENTED_EDGE('',*,*,#54844,.F.);
#78554=ORIENTED_EDGE('',*,*,#56325,.T.);
#78555=ORIENTED_EDGE('',*,*,#54846,.F.);
#78556=ORIENTED_EDGE('',*,*,#56326,.T.);
#78557=ORIENTED_EDGE('',*,*,#54850,.F.);
#78558=ORIENTED_EDGE('',*,*,#56327,.T.);
#78559=ORIENTED_EDGE('',*,*,#54890,.F.);
#78560=ORIENTED_EDGE('',*,*,#56328,.T.);
#78561=ORIENTED_EDGE('',*,*,#54872,.F.);
#78562=ORIENTED_EDGE('',*,*,#56329,.T.);
#78563=ORIENTED_EDGE('',*,*,#54874,.F.);
#78564=ORIENTED_EDGE('',*,*,#56330,.T.);
#78565=ORIENTED_EDGE('',*,*,#54878,.F.);
#78566=ORIENTED_EDGE('',*,*,#56331,.T.);
#78567=ORIENTED_EDGE('',*,*,#54918,.F.);
#78568=ORIENTED_EDGE('',*,*,#56332,.T.);
#78569=ORIENTED_EDGE('',*,*,#54900,.F.);
#78570=ORIENTED_EDGE('',*,*,#56333,.T.);
#78571=ORIENTED_EDGE('',*,*,#54902,.F.);
#78572=ORIENTED_EDGE('',*,*,#56334,.T.);
#78573=ORIENTED_EDGE('',*,*,#54906,.F.);
#78574=ORIENTED_EDGE('',*,*,#56335,.T.);
#78575=ORIENTED_EDGE('',*,*,#54946,.F.);
#78576=ORIENTED_EDGE('',*,*,#56336,.T.);
#78577=ORIENTED_EDGE('',*,*,#54928,.F.);
#78578=ORIENTED_EDGE('',*,*,#56337,.T.);
#78579=ORIENTED_EDGE('',*,*,#54930,.F.);
#78580=ORIENTED_EDGE('',*,*,#56338,.T.);
#78581=ORIENTED_EDGE('',*,*,#54934,.F.);
#78582=ORIENTED_EDGE('',*,*,#56339,.T.);
#78583=ORIENTED_EDGE('',*,*,#54974,.F.);
#78584=ORIENTED_EDGE('',*,*,#56340,.T.);
#78585=ORIENTED_EDGE('',*,*,#54956,.F.);
#78586=ORIENTED_EDGE('',*,*,#56341,.T.);
#78587=ORIENTED_EDGE('',*,*,#54958,.F.);
#78588=ORIENTED_EDGE('',*,*,#56342,.T.);
#78589=ORIENTED_EDGE('',*,*,#54962,.F.);
#78590=ORIENTED_EDGE('',*,*,#56343,.T.);
#78591=ORIENTED_EDGE('',*,*,#55002,.F.);
#78592=ORIENTED_EDGE('',*,*,#56344,.T.);
#78593=ORIENTED_EDGE('',*,*,#54984,.F.);
#78594=ORIENTED_EDGE('',*,*,#56345,.T.);
#78595=ORIENTED_EDGE('',*,*,#54986,.F.);
#78596=ORIENTED_EDGE('',*,*,#56346,.T.);
#78597=ORIENTED_EDGE('',*,*,#54990,.F.);
#78598=ORIENTED_EDGE('',*,*,#56347,.T.);
#78599=ORIENTED_EDGE('',*,*,#55030,.F.);
#78600=ORIENTED_EDGE('',*,*,#56348,.T.);
#78601=ORIENTED_EDGE('',*,*,#55012,.F.);
#78602=ORIENTED_EDGE('',*,*,#56349,.T.);
#78603=ORIENTED_EDGE('',*,*,#55014,.F.);
#78604=ORIENTED_EDGE('',*,*,#56350,.T.);
#78605=ORIENTED_EDGE('',*,*,#55018,.F.);
#78606=ORIENTED_EDGE('',*,*,#56351,.T.);
#78607=ORIENTED_EDGE('',*,*,#55058,.F.);
#78608=ORIENTED_EDGE('',*,*,#56352,.T.);
#78609=ORIENTED_EDGE('',*,*,#55040,.F.);
#78610=ORIENTED_EDGE('',*,*,#56353,.T.);
#78611=ORIENTED_EDGE('',*,*,#55042,.F.);
#78612=ORIENTED_EDGE('',*,*,#56354,.T.);
#78613=ORIENTED_EDGE('',*,*,#55046,.F.);
#78614=ORIENTED_EDGE('',*,*,#56355,.T.);
#78615=ORIENTED_EDGE('',*,*,#55086,.F.);
#78616=ORIENTED_EDGE('',*,*,#56356,.T.);
#78617=ORIENTED_EDGE('',*,*,#55068,.F.);
#78618=ORIENTED_EDGE('',*,*,#56357,.T.);
#78619=ORIENTED_EDGE('',*,*,#55070,.F.);
#78620=ORIENTED_EDGE('',*,*,#56358,.T.);
#78621=ORIENTED_EDGE('',*,*,#55074,.F.);
#78622=ORIENTED_EDGE('',*,*,#56359,.T.);
#78623=ORIENTED_EDGE('',*,*,#55114,.F.);
#78624=ORIENTED_EDGE('',*,*,#56360,.T.);
#78625=ORIENTED_EDGE('',*,*,#55096,.F.);
#78626=ORIENTED_EDGE('',*,*,#56361,.T.);
#78627=ORIENTED_EDGE('',*,*,#55098,.F.);
#78628=ORIENTED_EDGE('',*,*,#56362,.T.);
#78629=ORIENTED_EDGE('',*,*,#55102,.F.);
#78630=ORIENTED_EDGE('',*,*,#56363,.T.);
#78631=ORIENTED_EDGE('',*,*,#55142,.F.);
#78632=ORIENTED_EDGE('',*,*,#56364,.T.);
#78633=ORIENTED_EDGE('',*,*,#55124,.F.);
#78634=ORIENTED_EDGE('',*,*,#56365,.T.);
#78635=ORIENTED_EDGE('',*,*,#55126,.F.);
#78636=ORIENTED_EDGE('',*,*,#56366,.T.);
#78637=ORIENTED_EDGE('',*,*,#55130,.F.);
#78638=ORIENTED_EDGE('',*,*,#56367,.T.);
#78639=ORIENTED_EDGE('',*,*,#55170,.F.);
#78640=ORIENTED_EDGE('',*,*,#56368,.T.);
#78641=ORIENTED_EDGE('',*,*,#55152,.F.);
#78642=ORIENTED_EDGE('',*,*,#56369,.T.);
#78643=ORIENTED_EDGE('',*,*,#55154,.F.);
#78644=ORIENTED_EDGE('',*,*,#56370,.T.);
#78645=ORIENTED_EDGE('',*,*,#55158,.F.);
#78646=ORIENTED_EDGE('',*,*,#56371,.T.);
#78647=ORIENTED_EDGE('',*,*,#55198,.F.);
#78648=ORIENTED_EDGE('',*,*,#56372,.T.);
#78649=ORIENTED_EDGE('',*,*,#55180,.F.);
#78650=ORIENTED_EDGE('',*,*,#56373,.T.);
#78651=ORIENTED_EDGE('',*,*,#55182,.F.);
#78652=ORIENTED_EDGE('',*,*,#56374,.T.);
#78653=ORIENTED_EDGE('',*,*,#55186,.F.);
#78654=ORIENTED_EDGE('',*,*,#56375,.T.);
#78655=ORIENTED_EDGE('',*,*,#55226,.F.);
#78656=ORIENTED_EDGE('',*,*,#56376,.T.);
#78657=ORIENTED_EDGE('',*,*,#55208,.F.);
#78658=ORIENTED_EDGE('',*,*,#56377,.T.);
#78659=ORIENTED_EDGE('',*,*,#55210,.F.);
#78660=ORIENTED_EDGE('',*,*,#56378,.T.);
#78661=ORIENTED_EDGE('',*,*,#55214,.F.);
#78662=ORIENTED_EDGE('',*,*,#56379,.T.);
#78663=ORIENTED_EDGE('',*,*,#55254,.F.);
#78664=ORIENTED_EDGE('',*,*,#56380,.T.);
#78665=ORIENTED_EDGE('',*,*,#55236,.F.);
#78666=ORIENTED_EDGE('',*,*,#56381,.T.);
#78667=ORIENTED_EDGE('',*,*,#55238,.F.);
#78668=ORIENTED_EDGE('',*,*,#56382,.T.);
#78669=ORIENTED_EDGE('',*,*,#55242,.F.);
#78670=ORIENTED_EDGE('',*,*,#56383,.T.);
#78671=ORIENTED_EDGE('',*,*,#55282,.F.);
#78672=ORIENTED_EDGE('',*,*,#56384,.T.);
#78673=ORIENTED_EDGE('',*,*,#55264,.F.);
#78674=ORIENTED_EDGE('',*,*,#56385,.T.);
#78675=ORIENTED_EDGE('',*,*,#55266,.F.);
#78676=ORIENTED_EDGE('',*,*,#56386,.T.);
#78677=ORIENTED_EDGE('',*,*,#55270,.F.);
#78678=ORIENTED_EDGE('',*,*,#56387,.T.);
#78679=ORIENTED_EDGE('',*,*,#55310,.F.);
#78680=ORIENTED_EDGE('',*,*,#56388,.T.);
#78681=ORIENTED_EDGE('',*,*,#55292,.F.);
#78682=ORIENTED_EDGE('',*,*,#56389,.T.);
#78683=ORIENTED_EDGE('',*,*,#55294,.F.);
#78684=ORIENTED_EDGE('',*,*,#56390,.T.);
#78685=ORIENTED_EDGE('',*,*,#55298,.F.);
#78686=ORIENTED_EDGE('',*,*,#56391,.T.);
#78687=ORIENTED_EDGE('',*,*,#55338,.F.);
#78688=ORIENTED_EDGE('',*,*,#56392,.T.);
#78689=ORIENTED_EDGE('',*,*,#55320,.F.);
#78690=ORIENTED_EDGE('',*,*,#56393,.T.);
#78691=ORIENTED_EDGE('',*,*,#55322,.F.);
#78692=ORIENTED_EDGE('',*,*,#56394,.T.);
#78693=ORIENTED_EDGE('',*,*,#55326,.F.);
#78694=ORIENTED_EDGE('',*,*,#56395,.T.);
#78695=ORIENTED_EDGE('',*,*,#55366,.F.);
#78696=ORIENTED_EDGE('',*,*,#56396,.T.);
#78697=ORIENTED_EDGE('',*,*,#55348,.F.);
#78698=ORIENTED_EDGE('',*,*,#56397,.T.);
#78699=ORIENTED_EDGE('',*,*,#55350,.F.);
#78700=ORIENTED_EDGE('',*,*,#56398,.T.);
#78701=ORIENTED_EDGE('',*,*,#55354,.F.);
#78702=ORIENTED_EDGE('',*,*,#56399,.T.);
#78703=ORIENTED_EDGE('',*,*,#55394,.F.);
#78704=ORIENTED_EDGE('',*,*,#56400,.T.);
#78705=ORIENTED_EDGE('',*,*,#55376,.F.);
#78706=ORIENTED_EDGE('',*,*,#56401,.T.);
#78707=ORIENTED_EDGE('',*,*,#55378,.F.);
#78708=ORIENTED_EDGE('',*,*,#56402,.T.);
#78709=ORIENTED_EDGE('',*,*,#55382,.F.);
#78710=ORIENTED_EDGE('',*,*,#56403,.T.);
#78711=ORIENTED_EDGE('',*,*,#55422,.F.);
#78712=ORIENTED_EDGE('',*,*,#56404,.T.);
#78713=ORIENTED_EDGE('',*,*,#55404,.F.);
#78714=ORIENTED_EDGE('',*,*,#56405,.T.);
#78715=ORIENTED_EDGE('',*,*,#55406,.F.);
#78716=ORIENTED_EDGE('',*,*,#56406,.T.);
#78717=ORIENTED_EDGE('',*,*,#55410,.F.);
#78718=ORIENTED_EDGE('',*,*,#56407,.T.);
#78719=ORIENTED_EDGE('',*,*,#55450,.F.);
#78720=ORIENTED_EDGE('',*,*,#56408,.T.);
#78721=ORIENTED_EDGE('',*,*,#55432,.F.);
#78722=ORIENTED_EDGE('',*,*,#56409,.T.);
#78723=ORIENTED_EDGE('',*,*,#55434,.F.);
#78724=ORIENTED_EDGE('',*,*,#56410,.T.);
#78725=ORIENTED_EDGE('',*,*,#55438,.F.);
#78726=ORIENTED_EDGE('',*,*,#56411,.T.);
#78727=ORIENTED_EDGE('',*,*,#55476,.F.);
#78728=ORIENTED_EDGE('',*,*,#56412,.T.);
#78729=ORIENTED_EDGE('',*,*,#55460,.F.);
#78730=ORIENTED_EDGE('',*,*,#56413,.T.);
#78731=ORIENTED_EDGE('',*,*,#55461,.F.);
#78732=ORIENTED_EDGE('',*,*,#56414,.T.);
#78733=ORIENTED_EDGE('',*,*,#55464,.F.);
#78734=ORIENTED_EDGE('',*,*,#56415,.T.);
#78735=ORIENTED_EDGE('',*,*,#55504,.F.);
#78736=ORIENTED_EDGE('',*,*,#56416,.T.);
#78737=ORIENTED_EDGE('',*,*,#55486,.F.);
#78738=ORIENTED_EDGE('',*,*,#56417,.T.);
#78739=ORIENTED_EDGE('',*,*,#55488,.F.);
#78740=ORIENTED_EDGE('',*,*,#56418,.T.);
#78741=ORIENTED_EDGE('',*,*,#55492,.F.);
#78742=ORIENTED_EDGE('',*,*,#56419,.T.);
#78743=ORIENTED_EDGE('',*,*,#55532,.F.);
#78744=ORIENTED_EDGE('',*,*,#56420,.T.);
#78745=ORIENTED_EDGE('',*,*,#55514,.F.);
#78746=ORIENTED_EDGE('',*,*,#56421,.T.);
#78747=ORIENTED_EDGE('',*,*,#55516,.F.);
#78748=ORIENTED_EDGE('',*,*,#56422,.T.);
#78749=ORIENTED_EDGE('',*,*,#55520,.F.);
#78750=ORIENTED_EDGE('',*,*,#56423,.T.);
#78751=ORIENTED_EDGE('',*,*,#55560,.F.);
#78752=ORIENTED_EDGE('',*,*,#56424,.T.);
#78753=ORIENTED_EDGE('',*,*,#55542,.F.);
#78754=ORIENTED_EDGE('',*,*,#56425,.T.);
#78755=ORIENTED_EDGE('',*,*,#55544,.F.);
#78756=ORIENTED_EDGE('',*,*,#56426,.T.);
#78757=ORIENTED_EDGE('',*,*,#55548,.F.);
#78758=ORIENTED_EDGE('',*,*,#56427,.T.);
#78759=ORIENTED_EDGE('',*,*,#55588,.F.);
#78760=ORIENTED_EDGE('',*,*,#56428,.T.);
#78761=ORIENTED_EDGE('',*,*,#55570,.F.);
#78762=ORIENTED_EDGE('',*,*,#56429,.T.);
#78763=ORIENTED_EDGE('',*,*,#55572,.F.);
#78764=ORIENTED_EDGE('',*,*,#56430,.T.);
#78765=ORIENTED_EDGE('',*,*,#55576,.F.);
#78766=ORIENTED_EDGE('',*,*,#56431,.T.);
#78767=ORIENTED_EDGE('',*,*,#55616,.F.);
#78768=ORIENTED_EDGE('',*,*,#56432,.T.);
#78769=ORIENTED_EDGE('',*,*,#55598,.F.);
#78770=ORIENTED_EDGE('',*,*,#56433,.T.);
#78771=ORIENTED_EDGE('',*,*,#55600,.F.);
#78772=ORIENTED_EDGE('',*,*,#56434,.T.);
#78773=ORIENTED_EDGE('',*,*,#55604,.F.);
#78774=ORIENTED_EDGE('',*,*,#56435,.T.);
#78775=ORIENTED_EDGE('',*,*,#55644,.F.);
#78776=ORIENTED_EDGE('',*,*,#56436,.T.);
#78777=ORIENTED_EDGE('',*,*,#55626,.F.);
#78778=ORIENTED_EDGE('',*,*,#56437,.T.);
#78779=ORIENTED_EDGE('',*,*,#55628,.F.);
#78780=ORIENTED_EDGE('',*,*,#56438,.T.);
#78781=ORIENTED_EDGE('',*,*,#55632,.F.);
#78782=ORIENTED_EDGE('',*,*,#56439,.T.);
#78783=ORIENTED_EDGE('',*,*,#55672,.F.);
#78784=ORIENTED_EDGE('',*,*,#56440,.T.);
#78785=ORIENTED_EDGE('',*,*,#55654,.F.);
#78786=ORIENTED_EDGE('',*,*,#56441,.T.);
#78787=ORIENTED_EDGE('',*,*,#55656,.F.);
#78788=ORIENTED_EDGE('',*,*,#56442,.T.);
#78789=ORIENTED_EDGE('',*,*,#55660,.F.);
#78790=ORIENTED_EDGE('',*,*,#56443,.T.);
#78791=ORIENTED_EDGE('',*,*,#55700,.F.);
#78792=ORIENTED_EDGE('',*,*,#56444,.T.);
#78793=ORIENTED_EDGE('',*,*,#55682,.F.);
#78794=ORIENTED_EDGE('',*,*,#56445,.T.);
#78795=ORIENTED_EDGE('',*,*,#55684,.F.);
#78796=ORIENTED_EDGE('',*,*,#56446,.T.);
#78797=ORIENTED_EDGE('',*,*,#55688,.F.);
#78798=ORIENTED_EDGE('',*,*,#56447,.T.);
#78799=ORIENTED_EDGE('',*,*,#55728,.F.);
#78800=ORIENTED_EDGE('',*,*,#56448,.T.);
#78801=ORIENTED_EDGE('',*,*,#55710,.F.);
#78802=ORIENTED_EDGE('',*,*,#56449,.T.);
#78803=ORIENTED_EDGE('',*,*,#55712,.F.);
#78804=ORIENTED_EDGE('',*,*,#56450,.T.);
#78805=ORIENTED_EDGE('',*,*,#55716,.F.);
#78806=ORIENTED_EDGE('',*,*,#56451,.T.);
#78807=ORIENTED_EDGE('',*,*,#55756,.F.);
#78808=ORIENTED_EDGE('',*,*,#56452,.T.);
#78809=ORIENTED_EDGE('',*,*,#55738,.F.);
#78810=ORIENTED_EDGE('',*,*,#56453,.T.);
#78811=ORIENTED_EDGE('',*,*,#55740,.F.);
#78812=ORIENTED_EDGE('',*,*,#56454,.T.);
#78813=ORIENTED_EDGE('',*,*,#55744,.F.);
#78814=ORIENTED_EDGE('',*,*,#56455,.T.);
#78815=ORIENTED_EDGE('',*,*,#55784,.F.);
#78816=ORIENTED_EDGE('',*,*,#56456,.T.);
#78817=ORIENTED_EDGE('',*,*,#55766,.F.);
#78818=ORIENTED_EDGE('',*,*,#56457,.T.);
#78819=ORIENTED_EDGE('',*,*,#55768,.F.);
#78820=ORIENTED_EDGE('',*,*,#56458,.T.);
#78821=ORIENTED_EDGE('',*,*,#55772,.F.);
#78822=ORIENTED_EDGE('',*,*,#56459,.T.);
#78823=ORIENTED_EDGE('',*,*,#55812,.F.);
#78824=ORIENTED_EDGE('',*,*,#56460,.T.);
#78825=ORIENTED_EDGE('',*,*,#55794,.F.);
#78826=ORIENTED_EDGE('',*,*,#56461,.T.);
#78827=ORIENTED_EDGE('',*,*,#55796,.F.);
#78828=ORIENTED_EDGE('',*,*,#56462,.T.);
#78829=ORIENTED_EDGE('',*,*,#55800,.F.);
#78830=ORIENTED_EDGE('',*,*,#56463,.T.);
#78831=ORIENTED_EDGE('',*,*,#55840,.F.);
#78832=ORIENTED_EDGE('',*,*,#56464,.T.);
#78833=ORIENTED_EDGE('',*,*,#55822,.F.);
#78834=ORIENTED_EDGE('',*,*,#56465,.T.);
#78835=ORIENTED_EDGE('',*,*,#55824,.F.);
#78836=ORIENTED_EDGE('',*,*,#56466,.T.);
#78837=ORIENTED_EDGE('',*,*,#55828,.F.);
#78838=ORIENTED_EDGE('',*,*,#56467,.T.);
#78839=ORIENTED_EDGE('',*,*,#55868,.F.);
#78840=ORIENTED_EDGE('',*,*,#56468,.T.);
#78841=ORIENTED_EDGE('',*,*,#55850,.F.);
#78842=ORIENTED_EDGE('',*,*,#56469,.T.);
#78843=ORIENTED_EDGE('',*,*,#55852,.F.);
#78844=ORIENTED_EDGE('',*,*,#56470,.T.);
#78845=ORIENTED_EDGE('',*,*,#55856,.F.);
#78846=ORIENTED_EDGE('',*,*,#56471,.T.);
#78847=ORIENTED_EDGE('',*,*,#55894,.F.);
#78848=ORIENTED_EDGE('',*,*,#56472,.T.);
#78849=ORIENTED_EDGE('',*,*,#55878,.F.);
#78850=ORIENTED_EDGE('',*,*,#56473,.T.);
#78851=ORIENTED_EDGE('',*,*,#55879,.F.);
#78852=ORIENTED_EDGE('',*,*,#56474,.T.);
#78853=ORIENTED_EDGE('',*,*,#55882,.F.);
#78854=ORIENTED_EDGE('',*,*,#56475,.T.);
#78855=ORIENTED_EDGE('',*,*,#55922,.F.);
#78856=ORIENTED_EDGE('',*,*,#56476,.T.);
#78857=ORIENTED_EDGE('',*,*,#55904,.F.);
#78858=ORIENTED_EDGE('',*,*,#56477,.T.);
#78859=ORIENTED_EDGE('',*,*,#55906,.F.);
#78860=ORIENTED_EDGE('',*,*,#56478,.T.);
#78861=ORIENTED_EDGE('',*,*,#55910,.F.);
#78862=ORIENTED_EDGE('',*,*,#56479,.T.);
#78863=ORIENTED_EDGE('',*,*,#55950,.F.);
#78864=ORIENTED_EDGE('',*,*,#56480,.T.);
#78865=ORIENTED_EDGE('',*,*,#55932,.F.);
#78866=ORIENTED_EDGE('',*,*,#56481,.T.);
#78867=ORIENTED_EDGE('',*,*,#55934,.F.);
#78868=ORIENTED_EDGE('',*,*,#56482,.T.);
#78869=ORIENTED_EDGE('',*,*,#55938,.F.);
#78870=ORIENTED_EDGE('',*,*,#56483,.T.);
#78871=ORIENTED_EDGE('',*,*,#55978,.F.);
#78872=ORIENTED_EDGE('',*,*,#56484,.T.);
#78873=ORIENTED_EDGE('',*,*,#55960,.F.);
#78874=ORIENTED_EDGE('',*,*,#56485,.T.);
#78875=ORIENTED_EDGE('',*,*,#55962,.F.);
#78876=ORIENTED_EDGE('',*,*,#56486,.T.);
#78877=ORIENTED_EDGE('',*,*,#55966,.F.);
#78878=ORIENTED_EDGE('',*,*,#56487,.T.);
#78879=ORIENTED_EDGE('',*,*,#56006,.F.);
#78880=ORIENTED_EDGE('',*,*,#56488,.T.);
#78881=ORIENTED_EDGE('',*,*,#55988,.F.);
#78882=ORIENTED_EDGE('',*,*,#56489,.T.);
#78883=ORIENTED_EDGE('',*,*,#55990,.F.);
#78884=ORIENTED_EDGE('',*,*,#56490,.T.);
#78885=ORIENTED_EDGE('',*,*,#55994,.F.);
#78886=ORIENTED_EDGE('',*,*,#56491,.T.);
#78887=ORIENTED_EDGE('',*,*,#56034,.F.);
#78888=ORIENTED_EDGE('',*,*,#56492,.T.);
#78889=ORIENTED_EDGE('',*,*,#56016,.F.);
#78890=ORIENTED_EDGE('',*,*,#56493,.T.);
#78891=ORIENTED_EDGE('',*,*,#56018,.F.);
#78892=ORIENTED_EDGE('',*,*,#56494,.T.);
#78893=ORIENTED_EDGE('',*,*,#56022,.F.);
#78894=ORIENTED_EDGE('',*,*,#56495,.T.);
#78895=ORIENTED_EDGE('',*,*,#56062,.F.);
#78896=ORIENTED_EDGE('',*,*,#56496,.T.);
#78897=ORIENTED_EDGE('',*,*,#56044,.F.);
#78898=ORIENTED_EDGE('',*,*,#56497,.T.);
#78899=ORIENTED_EDGE('',*,*,#56046,.F.);
#78900=ORIENTED_EDGE('',*,*,#56498,.T.);
#78901=ORIENTED_EDGE('',*,*,#56050,.F.);
#78902=ORIENTED_EDGE('',*,*,#56499,.T.);
#78903=ORIENTED_EDGE('',*,*,#56090,.F.);
#78904=ORIENTED_EDGE('',*,*,#56500,.T.);
#78905=ORIENTED_EDGE('',*,*,#56072,.F.);
#78906=ORIENTED_EDGE('',*,*,#56501,.T.);
#78907=ORIENTED_EDGE('',*,*,#56074,.F.);
#78908=ORIENTED_EDGE('',*,*,#56502,.T.);
#78909=ORIENTED_EDGE('',*,*,#56078,.F.);
#78910=ORIENTED_EDGE('',*,*,#56503,.T.);
#78911=ORIENTED_EDGE('',*,*,#56118,.F.);
#78912=ORIENTED_EDGE('',*,*,#56504,.T.);
#78913=ORIENTED_EDGE('',*,*,#56100,.F.);
#78914=ORIENTED_EDGE('',*,*,#56505,.T.);
#78915=ORIENTED_EDGE('',*,*,#56102,.F.);
#78916=ORIENTED_EDGE('',*,*,#56506,.T.);
#78917=ORIENTED_EDGE('',*,*,#56106,.F.);
#78918=ORIENTED_EDGE('',*,*,#56507,.T.);
#78919=ORIENTED_EDGE('',*,*,#56146,.F.);
#78920=ORIENTED_EDGE('',*,*,#56508,.T.);
#78921=ORIENTED_EDGE('',*,*,#56128,.F.);
#78922=ORIENTED_EDGE('',*,*,#56509,.T.);
#78923=ORIENTED_EDGE('',*,*,#56130,.F.);
#78924=ORIENTED_EDGE('',*,*,#56510,.T.);
#78925=ORIENTED_EDGE('',*,*,#56134,.F.);
#78926=ORIENTED_EDGE('',*,*,#56511,.T.);
#78927=ORIENTED_EDGE('',*,*,#56174,.F.);
#78928=ORIENTED_EDGE('',*,*,#56512,.T.);
#78929=ORIENTED_EDGE('',*,*,#56156,.F.);
#78930=ORIENTED_EDGE('',*,*,#56513,.T.);
#78931=ORIENTED_EDGE('',*,*,#56158,.F.);
#78932=ORIENTED_EDGE('',*,*,#56514,.T.);
#78933=ORIENTED_EDGE('',*,*,#56162,.F.);
#78934=ORIENTED_EDGE('',*,*,#56515,.T.);
#78935=ORIENTED_EDGE('',*,*,#56202,.F.);
#78936=ORIENTED_EDGE('',*,*,#56516,.T.);
#78937=ORIENTED_EDGE('',*,*,#56184,.F.);
#78938=ORIENTED_EDGE('',*,*,#56517,.T.);
#78939=ORIENTED_EDGE('',*,*,#56186,.F.);
#78940=ORIENTED_EDGE('',*,*,#56518,.T.);
#78941=ORIENTED_EDGE('',*,*,#56190,.F.);
#78942=ORIENTED_EDGE('',*,*,#56519,.T.);
#78943=ORIENTED_EDGE('',*,*,#56230,.F.);
#78944=ORIENTED_EDGE('',*,*,#56520,.T.);
#78945=ORIENTED_EDGE('',*,*,#56212,.F.);
#78946=ORIENTED_EDGE('',*,*,#56521,.T.);
#78947=ORIENTED_EDGE('',*,*,#56214,.F.);
#78948=ORIENTED_EDGE('',*,*,#56522,.T.);
#78949=ORIENTED_EDGE('',*,*,#56218,.F.);
#78950=ORIENTED_EDGE('',*,*,#56523,.T.);
#78951=ORIENTED_EDGE('',*,*,#56258,.F.);
#78952=ORIENTED_EDGE('',*,*,#56524,.T.);
#78953=ORIENTED_EDGE('',*,*,#56240,.F.);
#78954=ORIENTED_EDGE('',*,*,#56525,.T.);
#78955=ORIENTED_EDGE('',*,*,#56242,.F.);
#78956=ORIENTED_EDGE('',*,*,#56526,.T.);
#78957=ORIENTED_EDGE('',*,*,#56246,.F.);
#78958=ORIENTED_EDGE('',*,*,#56527,.T.);
#78959=ORIENTED_EDGE('',*,*,#56286,.F.);
#78960=ORIENTED_EDGE('',*,*,#56528,.T.);
#78961=ORIENTED_EDGE('',*,*,#56268,.F.);
#78962=ORIENTED_EDGE('',*,*,#56529,.T.);
#78963=ORIENTED_EDGE('',*,*,#56270,.F.);
#78964=ORIENTED_EDGE('',*,*,#56530,.T.);
#78965=ORIENTED_EDGE('',*,*,#56274,.F.);
#78966=ORIENTED_EDGE('',*,*,#56531,.T.);
#78967=ORIENTED_EDGE('',*,*,#56532,.F.);
#78968=ORIENTED_EDGE('',*,*,#54674,.F.);
#78969=ORIENTED_EDGE('',*,*,#56533,.F.);
#78970=ORIENTED_EDGE('',*,*,#54546,.F.);
#78971=ORIENTED_EDGE('',*,*,#56533,.T.);
#78972=ORIENTED_EDGE('',*,*,#54673,.F.);
#78973=ORIENTED_EDGE('',*,*,#56534,.F.);
#78974=ORIENTED_EDGE('',*,*,#54555,.F.);
#78975=ORIENTED_EDGE('',*,*,#54545,.T.);
#78976=ORIENTED_EDGE('',*,*,#54549,.F.);
#78977=ORIENTED_EDGE('',*,*,#56535,.F.);
#78978=ORIENTED_EDGE('',*,*,#54675,.F.);
#78979=ORIENTED_EDGE('',*,*,#56532,.T.);
#78980=ORIENTED_EDGE('',*,*,#56534,.T.);
#78981=ORIENTED_EDGE('',*,*,#54672,.F.);
#78982=ORIENTED_EDGE('',*,*,#56536,.F.);
#78983=ORIENTED_EDGE('',*,*,#54540,.F.);
#78984=ORIENTED_EDGE('',*,*,#56535,.T.);
#78985=ORIENTED_EDGE('',*,*,#54553,.F.);
#78986=ORIENTED_EDGE('',*,*,#56537,.F.);
#78987=ORIENTED_EDGE('',*,*,#54664,.F.);
#78988=ORIENTED_EDGE('',*,*,#56536,.T.);
#78989=ORIENTED_EDGE('',*,*,#54671,.F.);
#78990=ORIENTED_EDGE('',*,*,#56538,.F.);
#78991=ORIENTED_EDGE('',*,*,#54557,.F.);
#78992=ORIENTED_EDGE('',*,*,#56537,.T.);
#78993=ORIENTED_EDGE('',*,*,#52072,.F.);
#78994=ORIENTED_EDGE('',*,*,#56539,.F.);
#78995=ORIENTED_EDGE('',*,*,#54665,.F.);
#78996=ORIENTED_EDGE('',*,*,#56538,.T.);
#78997=ORIENTED_EDGE('',*,*,#54670,.F.);
#78998=ORIENTED_EDGE('',*,*,#56540,.F.);
#78999=ORIENTED_EDGE('',*,*,#54532,.T.);
#79000=ORIENTED_EDGE('',*,*,#54536,.F.);
#79001=ORIENTED_EDGE('',*,*,#56539,.T.);
#79002=ORIENTED_EDGE('',*,*,#52071,.F.);
#79003=ORIENTED_EDGE('',*,*,#56541,.F.);
#79004=ORIENTED_EDGE('',*,*,#56296,.F.);
#79005=ORIENTED_EDGE('',*,*,#56540,.T.);
#79006=ORIENTED_EDGE('',*,*,#54669,.F.);
#79007=ORIENTED_EDGE('',*,*,#56542,.F.);
#79008=ORIENTED_EDGE('',*,*,#54533,.F.);
#79009=ORIENTED_EDGE('',*,*,#56541,.T.);
#79010=ORIENTED_EDGE('',*,*,#52070,.F.);
#79011=ORIENTED_EDGE('',*,*,#56543,.F.);
#79012=ORIENTED_EDGE('',*,*,#54649,.F.);
#79013=ORIENTED_EDGE('',*,*,#56542,.T.);
#79014=ORIENTED_EDGE('',*,*,#54668,.F.);
#79015=ORIENTED_EDGE('',*,*,#56544,.F.);
#79016=ORIENTED_EDGE('',*,*,#54551,.F.);
#79017=ORIENTED_EDGE('',*,*,#56543,.T.);
#79018=ORIENTED_EDGE('',*,*,#52069,.F.);
#79019=ORIENTED_EDGE('',*,*,#56545,.F.);
#79020=ORIENTED_EDGE('',*,*,#56298,.F.);
#79021=ORIENTED_EDGE('',*,*,#56544,.T.);
#79022=ORIENTED_EDGE('',*,*,#54667,.F.);
#79023=ORIENTED_EDGE('',*,*,#56546,.F.);
#79024=ORIENTED_EDGE('',*,*,#52594,.F.);
#79025=ORIENTED_EDGE('',*,*,#56545,.T.);
#79026=ORIENTED_EDGE('',*,*,#52068,.F.);
#79027=ORIENTED_EDGE('',*,*,#56547,.F.);
#79028=ORIENTED_EDGE('',*,*,#54655,.F.);
#79029=ORIENTED_EDGE('',*,*,#56546,.T.);
#79030=ORIENTED_EDGE('',*,*,#56297,.F.);
#79031=ORIENTED_EDGE('',*,*,#56548,.F.);
#79032=ORIENTED_EDGE('',*,*,#52595,.F.);
#79033=ORIENTED_EDGE('',*,*,#56547,.T.);
#79034=ORIENTED_EDGE('',*,*,#54582,.F.);
#79035=ORIENTED_EDGE('',*,*,#56549,.F.);
#79036=ORIENTED_EDGE('',*,*,#54656,.F.);
#79037=ORIENTED_EDGE('',*,*,#56548,.T.);
#79038=ORIENTED_EDGE('',*,*,#54651,.F.);
#79039=ORIENTED_EDGE('',*,*,#56550,.F.);
#79040=ORIENTED_EDGE('',*,*,#52596,.F.);
#79041=ORIENTED_EDGE('',*,*,#54577,.F.);
#79042=ORIENTED_EDGE('',*,*,#54573,.T.);
#79043=ORIENTED_EDGE('',*,*,#56551,.F.);
#79044=ORIENTED_EDGE('',*,*,#54657,.F.);
#79045=ORIENTED_EDGE('',*,*,#56549,.T.);
#79046=ORIENTED_EDGE('',*,*,#56550,.T.);
#79047=ORIENTED_EDGE('',*,*,#56299,.F.);
#79048=ORIENTED_EDGE('',*,*,#56552,.F.);
#79049=ORIENTED_EDGE('',*,*,#52597,.F.);
#79050=ORIENTED_EDGE('',*,*,#56551,.T.);
#79051=ORIENTED_EDGE('',*,*,#54572,.F.);
#79052=ORIENTED_EDGE('',*,*,#56553,.F.);
#79053=ORIENTED_EDGE('',*,*,#54658,.F.);
#79054=ORIENTED_EDGE('',*,*,#56552,.T.);
#79055=ORIENTED_EDGE('',*,*,#54653,.F.);
#79056=ORIENTED_EDGE('',*,*,#56554,.F.);
#79057=ORIENTED_EDGE('',*,*,#52598,.F.);
#79058=ORIENTED_EDGE('',*,*,#56553,.T.);
#79059=ORIENTED_EDGE('',*,*,#54584,.F.);
#79060=ORIENTED_EDGE('',*,*,#56555,.F.);
#79061=ORIENTED_EDGE('',*,*,#54659,.F.);
#79062=ORIENTED_EDGE('',*,*,#56554,.T.);
#79063=ORIENTED_EDGE('',*,*,#54652,.F.);
#79064=ORIENTED_EDGE('',*,*,#56556,.F.);
#79065=ORIENTED_EDGE('',*,*,#54580,.F.);
#79066=ORIENTED_EDGE('',*,*,#56555,.T.);
#79067=ORIENTED_EDGE('',*,*,#54568,.F.);
#79068=ORIENTED_EDGE('',*,*,#56557,.F.);
#79069=ORIENTED_EDGE('',*,*,#54660,.F.);
#79070=ORIENTED_EDGE('',*,*,#56556,.T.);
#79071=ORIENTED_EDGE('',*,*,#54663,.F.);
#79072=ORIENTED_EDGE('',*,*,#56558,.F.);
#79073=ORIENTED_EDGE('',*,*,#54559,.F.);
#79074=ORIENTED_EDGE('',*,*,#56557,.T.);
#79075=ORIENTED_EDGE('',*,*,#54586,.F.);
#79076=ORIENTED_EDGE('',*,*,#56559,.F.);
#79077=ORIENTED_EDGE('',*,*,#54661,.F.);
#79078=ORIENTED_EDGE('',*,*,#56558,.T.);
#79079=ORIENTED_EDGE('',*,*,#54662,.F.);
#79080=ORIENTED_EDGE('',*,*,#56559,.T.);
#79081=ORIENTED_EDGE('',*,*,#54564,.F.);
#79082=ORIENTED_EDGE('',*,*,#54560,.T.);
#79083=ORIENTED_EDGE('',*,*,#56560,.F.);
#79084=ORIENTED_EDGE('',*,*,#54702,.F.);
#79085=ORIENTED_EDGE('',*,*,#56561,.F.);
#79086=ORIENTED_EDGE('',*,*,#54516,.F.);
#79087=ORIENTED_EDGE('',*,*,#56561,.T.);
#79088=ORIENTED_EDGE('',*,*,#54701,.F.);
#79089=ORIENTED_EDGE('',*,*,#56562,.F.);
#79090=ORIENTED_EDGE('',*,*,#54525,.F.);
#79091=ORIENTED_EDGE('',*,*,#54515,.T.);
#79092=ORIENTED_EDGE('',*,*,#54519,.F.);
#79093=ORIENTED_EDGE('',*,*,#56563,.F.);
#79094=ORIENTED_EDGE('',*,*,#54703,.F.);
#79095=ORIENTED_EDGE('',*,*,#56560,.T.);
#79096=ORIENTED_EDGE('',*,*,#56562,.T.);
#79097=ORIENTED_EDGE('',*,*,#54700,.F.);
#79098=ORIENTED_EDGE('',*,*,#56564,.F.);
#79099=ORIENTED_EDGE('',*,*,#54510,.F.);
#79100=ORIENTED_EDGE('',*,*,#56563,.T.);
#79101=ORIENTED_EDGE('',*,*,#54523,.F.);
#79102=ORIENTED_EDGE('',*,*,#56565,.F.);
#79103=ORIENTED_EDGE('',*,*,#54692,.F.);
#79104=ORIENTED_EDGE('',*,*,#56564,.T.);
#79105=ORIENTED_EDGE('',*,*,#54699,.F.);
#79106=ORIENTED_EDGE('',*,*,#56566,.F.);
#79107=ORIENTED_EDGE('',*,*,#54527,.F.);
#79108=ORIENTED_EDGE('',*,*,#56565,.T.);
#79109=ORIENTED_EDGE('',*,*,#52078,.F.);
#79110=ORIENTED_EDGE('',*,*,#56567,.F.);
#79111=ORIENTED_EDGE('',*,*,#54693,.F.);
#79112=ORIENTED_EDGE('',*,*,#56566,.T.);
#79113=ORIENTED_EDGE('',*,*,#54698,.F.);
#79114=ORIENTED_EDGE('',*,*,#56568,.F.);
#79115=ORIENTED_EDGE('',*,*,#54502,.T.);
#79116=ORIENTED_EDGE('',*,*,#54506,.F.);
#79117=ORIENTED_EDGE('',*,*,#56567,.T.);
#79118=ORIENTED_EDGE('',*,*,#52077,.F.);
#79119=ORIENTED_EDGE('',*,*,#56569,.F.);
#79120=ORIENTED_EDGE('',*,*,#56300,.F.);
#79121=ORIENTED_EDGE('',*,*,#56568,.T.);
#79122=ORIENTED_EDGE('',*,*,#54697,.F.);
#79123=ORIENTED_EDGE('',*,*,#56570,.F.);
#79124=ORIENTED_EDGE('',*,*,#54503,.F.);
#79125=ORIENTED_EDGE('',*,*,#56569,.T.);
#79126=ORIENTED_EDGE('',*,*,#52076,.F.);
#79127=ORIENTED_EDGE('',*,*,#56571,.F.);
#79128=ORIENTED_EDGE('',*,*,#54677,.F.);
#79129=ORIENTED_EDGE('',*,*,#56570,.T.);
#79130=ORIENTED_EDGE('',*,*,#54696,.F.);
#79131=ORIENTED_EDGE('',*,*,#56572,.F.);
#79132=ORIENTED_EDGE('',*,*,#54521,.F.);
#79133=ORIENTED_EDGE('',*,*,#56571,.T.);
#79134=ORIENTED_EDGE('',*,*,#52075,.F.);
#79135=ORIENTED_EDGE('',*,*,#56573,.F.);
#79136=ORIENTED_EDGE('',*,*,#56302,.F.);
#79137=ORIENTED_EDGE('',*,*,#56572,.T.);
#79138=ORIENTED_EDGE('',*,*,#54695,.F.);
#79139=ORIENTED_EDGE('',*,*,#56574,.F.);
#79140=ORIENTED_EDGE('',*,*,#52588,.F.);
#79141=ORIENTED_EDGE('',*,*,#56573,.T.);
#79142=ORIENTED_EDGE('',*,*,#52074,.F.);
#79143=ORIENTED_EDGE('',*,*,#56575,.F.);
#79144=ORIENTED_EDGE('',*,*,#54683,.F.);
#79145=ORIENTED_EDGE('',*,*,#56574,.T.);
#79146=ORIENTED_EDGE('',*,*,#56301,.F.);
#79147=ORIENTED_EDGE('',*,*,#56576,.F.);
#79148=ORIENTED_EDGE('',*,*,#52589,.F.);
#79149=ORIENTED_EDGE('',*,*,#56575,.T.);
#79150=ORIENTED_EDGE('',*,*,#54552,.F.);
#79151=ORIENTED_EDGE('',*,*,#56577,.F.);
#79152=ORIENTED_EDGE('',*,*,#54684,.F.);
#79153=ORIENTED_EDGE('',*,*,#56576,.T.);
#79154=ORIENTED_EDGE('',*,*,#54679,.F.);
#79155=ORIENTED_EDGE('',*,*,#56578,.F.);
#79156=ORIENTED_EDGE('',*,*,#52590,.F.);
#79157=ORIENTED_EDGE('',*,*,#54547,.F.);
#79158=ORIENTED_EDGE('',*,*,#54543,.T.);
#79159=ORIENTED_EDGE('',*,*,#56579,.F.);
#79160=ORIENTED_EDGE('',*,*,#54685,.F.);
#79161=ORIENTED_EDGE('',*,*,#56577,.T.);
#79162=ORIENTED_EDGE('',*,*,#56578,.T.);
#79163=ORIENTED_EDGE('',*,*,#56303,.F.);
#79164=ORIENTED_EDGE('',*,*,#56580,.F.);
#79165=ORIENTED_EDGE('',*,*,#52591,.F.);
#79166=ORIENTED_EDGE('',*,*,#56579,.T.);
#79167=ORIENTED_EDGE('',*,*,#54542,.F.);
#79168=ORIENTED_EDGE('',*,*,#56581,.F.);
#79169=ORIENTED_EDGE('',*,*,#54686,.F.);
#79170=ORIENTED_EDGE('',*,*,#56580,.T.);
#79171=ORIENTED_EDGE('',*,*,#54681,.F.);
#79172=ORIENTED_EDGE('',*,*,#56582,.F.);
#79173=ORIENTED_EDGE('',*,*,#52592,.F.);
#79174=ORIENTED_EDGE('',*,*,#56581,.T.);
#79175=ORIENTED_EDGE('',*,*,#54554,.F.);
#79176=ORIENTED_EDGE('',*,*,#56583,.F.);
#79177=ORIENTED_EDGE('',*,*,#54687,.F.);
#79178=ORIENTED_EDGE('',*,*,#56582,.T.);
#79179=ORIENTED_EDGE('',*,*,#54680,.F.);
#79180=ORIENTED_EDGE('',*,*,#56584,.F.);
#79181=ORIENTED_EDGE('',*,*,#54550,.F.);
#79182=ORIENTED_EDGE('',*,*,#56583,.T.);
#79183=ORIENTED_EDGE('',*,*,#54538,.F.);
#79184=ORIENTED_EDGE('',*,*,#56585,.F.);
#79185=ORIENTED_EDGE('',*,*,#54688,.F.);
#79186=ORIENTED_EDGE('',*,*,#56584,.T.);
#79187=ORIENTED_EDGE('',*,*,#54691,.F.);
#79188=ORIENTED_EDGE('',*,*,#56586,.F.);
#79189=ORIENTED_EDGE('',*,*,#54529,.F.);
#79190=ORIENTED_EDGE('',*,*,#56585,.T.);
#79191=ORIENTED_EDGE('',*,*,#54556,.F.);
#79192=ORIENTED_EDGE('',*,*,#56587,.F.);
#79193=ORIENTED_EDGE('',*,*,#54689,.F.);
#79194=ORIENTED_EDGE('',*,*,#56586,.T.);
#79195=ORIENTED_EDGE('',*,*,#54690,.F.);
#79196=ORIENTED_EDGE('',*,*,#56587,.T.);
#79197=ORIENTED_EDGE('',*,*,#54534,.F.);
#79198=ORIENTED_EDGE('',*,*,#54530,.T.);
#79199=ORIENTED_EDGE('',*,*,#56588,.F.);
#79200=ORIENTED_EDGE('',*,*,#54730,.F.);
#79201=ORIENTED_EDGE('',*,*,#56589,.F.);
#79202=ORIENTED_EDGE('',*,*,#54486,.F.);
#79203=ORIENTED_EDGE('',*,*,#56589,.T.);
#79204=ORIENTED_EDGE('',*,*,#54729,.F.);
#79205=ORIENTED_EDGE('',*,*,#56590,.F.);
#79206=ORIENTED_EDGE('',*,*,#54495,.F.);
#79207=ORIENTED_EDGE('',*,*,#54485,.T.);
#79208=ORIENTED_EDGE('',*,*,#54489,.F.);
#79209=ORIENTED_EDGE('',*,*,#56591,.F.);
#79210=ORIENTED_EDGE('',*,*,#54731,.F.);
#79211=ORIENTED_EDGE('',*,*,#56588,.T.);
#79212=ORIENTED_EDGE('',*,*,#56590,.T.);
#79213=ORIENTED_EDGE('',*,*,#54728,.F.);
#79214=ORIENTED_EDGE('',*,*,#56592,.F.);
#79215=ORIENTED_EDGE('',*,*,#54480,.F.);
#79216=ORIENTED_EDGE('',*,*,#56591,.T.);
#79217=ORIENTED_EDGE('',*,*,#54493,.F.);
#79218=ORIENTED_EDGE('',*,*,#56593,.F.);
#79219=ORIENTED_EDGE('',*,*,#54720,.F.);
#79220=ORIENTED_EDGE('',*,*,#56592,.T.);
#79221=ORIENTED_EDGE('',*,*,#54727,.F.);
#79222=ORIENTED_EDGE('',*,*,#56594,.F.);
#79223=ORIENTED_EDGE('',*,*,#54497,.F.);
#79224=ORIENTED_EDGE('',*,*,#56593,.T.);
#79225=ORIENTED_EDGE('',*,*,#52084,.F.);
#79226=ORIENTED_EDGE('',*,*,#56595,.F.);
#79227=ORIENTED_EDGE('',*,*,#54721,.F.);
#79228=ORIENTED_EDGE('',*,*,#56594,.T.);
#79229=ORIENTED_EDGE('',*,*,#54726,.F.);
#79230=ORIENTED_EDGE('',*,*,#56596,.F.);
#79231=ORIENTED_EDGE('',*,*,#54472,.T.);
#79232=ORIENTED_EDGE('',*,*,#54476,.F.);
#79233=ORIENTED_EDGE('',*,*,#56595,.T.);
#79234=ORIENTED_EDGE('',*,*,#52083,.F.);
#79235=ORIENTED_EDGE('',*,*,#56597,.F.);
#79236=ORIENTED_EDGE('',*,*,#56304,.F.);
#79237=ORIENTED_EDGE('',*,*,#56596,.T.);
#79238=ORIENTED_EDGE('',*,*,#54725,.F.);
#79239=ORIENTED_EDGE('',*,*,#56598,.F.);
#79240=ORIENTED_EDGE('',*,*,#54473,.F.);
#79241=ORIENTED_EDGE('',*,*,#56597,.T.);
#79242=ORIENTED_EDGE('',*,*,#52082,.F.);
#79243=ORIENTED_EDGE('',*,*,#56599,.F.);
#79244=ORIENTED_EDGE('',*,*,#54705,.F.);
#79245=ORIENTED_EDGE('',*,*,#56598,.T.);
#79246=ORIENTED_EDGE('',*,*,#54724,.F.);
#79247=ORIENTED_EDGE('',*,*,#56600,.F.);
#79248=ORIENTED_EDGE('',*,*,#54491,.F.);
#79249=ORIENTED_EDGE('',*,*,#56599,.T.);
#79250=ORIENTED_EDGE('',*,*,#52081,.F.);
#79251=ORIENTED_EDGE('',*,*,#56601,.F.);
#79252=ORIENTED_EDGE('',*,*,#56306,.F.);
#79253=ORIENTED_EDGE('',*,*,#56600,.T.);
#79254=ORIENTED_EDGE('',*,*,#54723,.F.);
#79255=ORIENTED_EDGE('',*,*,#56602,.F.);
#79256=ORIENTED_EDGE('',*,*,#52582,.F.);
#79257=ORIENTED_EDGE('',*,*,#56601,.T.);
#79258=ORIENTED_EDGE('',*,*,#52080,.F.);
#79259=ORIENTED_EDGE('',*,*,#56603,.F.);
#79260=ORIENTED_EDGE('',*,*,#54711,.F.);
#79261=ORIENTED_EDGE('',*,*,#56602,.T.);
#79262=ORIENTED_EDGE('',*,*,#56305,.F.);
#79263=ORIENTED_EDGE('',*,*,#56604,.F.);
#79264=ORIENTED_EDGE('',*,*,#52583,.F.);
#79265=ORIENTED_EDGE('',*,*,#56603,.T.);
#79266=ORIENTED_EDGE('',*,*,#54522,.F.);
#79267=ORIENTED_EDGE('',*,*,#56605,.F.);
#79268=ORIENTED_EDGE('',*,*,#54712,.F.);
#79269=ORIENTED_EDGE('',*,*,#56604,.T.);
#79270=ORIENTED_EDGE('',*,*,#54707,.F.);
#79271=ORIENTED_EDGE('',*,*,#56606,.F.);
#79272=ORIENTED_EDGE('',*,*,#52584,.F.);
#79273=ORIENTED_EDGE('',*,*,#54517,.F.);
#79274=ORIENTED_EDGE('',*,*,#54513,.T.);
#79275=ORIENTED_EDGE('',*,*,#56607,.F.);
#79276=ORIENTED_EDGE('',*,*,#54713,.F.);
#79277=ORIENTED_EDGE('',*,*,#56605,.T.);
#79278=ORIENTED_EDGE('',*,*,#56606,.T.);
#79279=ORIENTED_EDGE('',*,*,#56307,.F.);
#79280=ORIENTED_EDGE('',*,*,#56608,.F.);
#79281=ORIENTED_EDGE('',*,*,#52585,.F.);
#79282=ORIENTED_EDGE('',*,*,#56607,.T.);
#79283=ORIENTED_EDGE('',*,*,#54512,.F.);
#79284=ORIENTED_EDGE('',*,*,#56609,.F.);
#79285=ORIENTED_EDGE('',*,*,#54714,.F.);
#79286=ORIENTED_EDGE('',*,*,#56608,.T.);
#79287=ORIENTED_EDGE('',*,*,#54709,.F.);
#79288=ORIENTED_EDGE('',*,*,#56610,.F.);
#79289=ORIENTED_EDGE('',*,*,#52586,.F.);
#79290=ORIENTED_EDGE('',*,*,#56609,.T.);
#79291=ORIENTED_EDGE('',*,*,#54524,.F.);
#79292=ORIENTED_EDGE('',*,*,#56611,.F.);
#79293=ORIENTED_EDGE('',*,*,#54715,.F.);
#79294=ORIENTED_EDGE('',*,*,#56610,.T.);
#79295=ORIENTED_EDGE('',*,*,#54708,.F.);
#79296=ORIENTED_EDGE('',*,*,#56612,.F.);
#79297=ORIENTED_EDGE('',*,*,#54520,.F.);
#79298=ORIENTED_EDGE('',*,*,#56611,.T.);
#79299=ORIENTED_EDGE('',*,*,#54508,.F.);
#79300=ORIENTED_EDGE('',*,*,#56613,.F.);
#79301=ORIENTED_EDGE('',*,*,#54716,.F.);
#79302=ORIENTED_EDGE('',*,*,#56612,.T.);
#79303=ORIENTED_EDGE('',*,*,#54719,.F.);
#79304=ORIENTED_EDGE('',*,*,#56614,.F.);
#79305=ORIENTED_EDGE('',*,*,#54499,.F.);
#79306=ORIENTED_EDGE('',*,*,#56613,.T.);
#79307=ORIENTED_EDGE('',*,*,#54526,.F.);
#79308=ORIENTED_EDGE('',*,*,#56615,.F.);
#79309=ORIENTED_EDGE('',*,*,#54717,.F.);
#79310=ORIENTED_EDGE('',*,*,#56614,.T.);
#79311=ORIENTED_EDGE('',*,*,#54718,.F.);
#79312=ORIENTED_EDGE('',*,*,#56615,.T.);
#79313=ORIENTED_EDGE('',*,*,#54504,.F.);
#79314=ORIENTED_EDGE('',*,*,#54500,.T.);
#79315=ORIENTED_EDGE('',*,*,#56616,.F.);
#79316=ORIENTED_EDGE('',*,*,#54758,.F.);
#79317=ORIENTED_EDGE('',*,*,#56617,.F.);
#79318=ORIENTED_EDGE('',*,*,#54456,.F.);
#79319=ORIENTED_EDGE('',*,*,#56617,.T.);
#79320=ORIENTED_EDGE('',*,*,#54757,.F.);
#79321=ORIENTED_EDGE('',*,*,#56618,.F.);
#79322=ORIENTED_EDGE('',*,*,#54465,.F.);
#79323=ORIENTED_EDGE('',*,*,#54455,.T.);
#79324=ORIENTED_EDGE('',*,*,#54459,.F.);
#79325=ORIENTED_EDGE('',*,*,#56619,.F.);
#79326=ORIENTED_EDGE('',*,*,#54759,.F.);
#79327=ORIENTED_EDGE('',*,*,#56616,.T.);
#79328=ORIENTED_EDGE('',*,*,#56618,.T.);
#79329=ORIENTED_EDGE('',*,*,#54756,.F.);
#79330=ORIENTED_EDGE('',*,*,#56620,.F.);
#79331=ORIENTED_EDGE('',*,*,#54450,.F.);
#79332=ORIENTED_EDGE('',*,*,#56619,.T.);
#79333=ORIENTED_EDGE('',*,*,#54463,.F.);
#79334=ORIENTED_EDGE('',*,*,#56621,.F.);
#79335=ORIENTED_EDGE('',*,*,#54748,.F.);
#79336=ORIENTED_EDGE('',*,*,#56620,.T.);
#79337=ORIENTED_EDGE('',*,*,#54755,.F.);
#79338=ORIENTED_EDGE('',*,*,#56622,.F.);
#79339=ORIENTED_EDGE('',*,*,#54467,.F.);
#79340=ORIENTED_EDGE('',*,*,#56621,.T.);
#79341=ORIENTED_EDGE('',*,*,#52090,.F.);
#79342=ORIENTED_EDGE('',*,*,#56623,.F.);
#79343=ORIENTED_EDGE('',*,*,#54749,.F.);
#79344=ORIENTED_EDGE('',*,*,#56622,.T.);
#79345=ORIENTED_EDGE('',*,*,#54754,.F.);
#79346=ORIENTED_EDGE('',*,*,#56624,.F.);
#79347=ORIENTED_EDGE('',*,*,#54442,.T.);
#79348=ORIENTED_EDGE('',*,*,#54446,.F.);
#79349=ORIENTED_EDGE('',*,*,#56623,.T.);
#79350=ORIENTED_EDGE('',*,*,#52089,.F.);
#79351=ORIENTED_EDGE('',*,*,#56625,.F.);
#79352=ORIENTED_EDGE('',*,*,#56308,.F.);
#79353=ORIENTED_EDGE('',*,*,#56624,.T.);
#79354=ORIENTED_EDGE('',*,*,#54753,.F.);
#79355=ORIENTED_EDGE('',*,*,#56626,.F.);
#79356=ORIENTED_EDGE('',*,*,#54443,.F.);
#79357=ORIENTED_EDGE('',*,*,#56625,.T.);
#79358=ORIENTED_EDGE('',*,*,#52088,.F.);
#79359=ORIENTED_EDGE('',*,*,#56627,.F.);
#79360=ORIENTED_EDGE('',*,*,#54733,.F.);
#79361=ORIENTED_EDGE('',*,*,#56626,.T.);
#79362=ORIENTED_EDGE('',*,*,#54752,.F.);
#79363=ORIENTED_EDGE('',*,*,#56628,.F.);
#79364=ORIENTED_EDGE('',*,*,#54461,.F.);
#79365=ORIENTED_EDGE('',*,*,#56627,.T.);
#79366=ORIENTED_EDGE('',*,*,#52087,.F.);
#79367=ORIENTED_EDGE('',*,*,#56629,.F.);
#79368=ORIENTED_EDGE('',*,*,#56310,.F.);
#79369=ORIENTED_EDGE('',*,*,#56628,.T.);
#79370=ORIENTED_EDGE('',*,*,#54751,.F.);
#79371=ORIENTED_EDGE('',*,*,#56630,.F.);
#79372=ORIENTED_EDGE('',*,*,#52576,.F.);
#79373=ORIENTED_EDGE('',*,*,#56629,.T.);
#79374=ORIENTED_EDGE('',*,*,#52086,.F.);
#79375=ORIENTED_EDGE('',*,*,#56631,.F.);
#79376=ORIENTED_EDGE('',*,*,#54739,.F.);
#79377=ORIENTED_EDGE('',*,*,#56630,.T.);
#79378=ORIENTED_EDGE('',*,*,#56309,.F.);
#79379=ORIENTED_EDGE('',*,*,#56632,.F.);
#79380=ORIENTED_EDGE('',*,*,#52577,.F.);
#79381=ORIENTED_EDGE('',*,*,#56631,.T.);
#79382=ORIENTED_EDGE('',*,*,#54492,.F.);
#79383=ORIENTED_EDGE('',*,*,#56633,.F.);
#79384=ORIENTED_EDGE('',*,*,#54740,.F.);
#79385=ORIENTED_EDGE('',*,*,#56632,.T.);
#79386=ORIENTED_EDGE('',*,*,#54735,.F.);
#79387=ORIENTED_EDGE('',*,*,#56634,.F.);
#79388=ORIENTED_EDGE('',*,*,#52578,.F.);
#79389=ORIENTED_EDGE('',*,*,#54487,.F.);
#79390=ORIENTED_EDGE('',*,*,#54483,.T.);
#79391=ORIENTED_EDGE('',*,*,#56635,.F.);
#79392=ORIENTED_EDGE('',*,*,#54741,.F.);
#79393=ORIENTED_EDGE('',*,*,#56633,.T.);
#79394=ORIENTED_EDGE('',*,*,#56634,.T.);
#79395=ORIENTED_EDGE('',*,*,#56311,.F.);
#79396=ORIENTED_EDGE('',*,*,#56636,.F.);
#79397=ORIENTED_EDGE('',*,*,#52579,.F.);
#79398=ORIENTED_EDGE('',*,*,#56635,.T.);
#79399=ORIENTED_EDGE('',*,*,#54482,.F.);
#79400=ORIENTED_EDGE('',*,*,#56637,.F.);
#79401=ORIENTED_EDGE('',*,*,#54742,.F.);
#79402=ORIENTED_EDGE('',*,*,#56636,.T.);
#79403=ORIENTED_EDGE('',*,*,#54737,.F.);
#79404=ORIENTED_EDGE('',*,*,#56638,.F.);
#79405=ORIENTED_EDGE('',*,*,#52580,.F.);
#79406=ORIENTED_EDGE('',*,*,#56637,.T.);
#79407=ORIENTED_EDGE('',*,*,#54494,.F.);
#79408=ORIENTED_EDGE('',*,*,#56639,.F.);
#79409=ORIENTED_EDGE('',*,*,#54743,.F.);
#79410=ORIENTED_EDGE('',*,*,#56638,.T.);
#79411=ORIENTED_EDGE('',*,*,#54736,.F.);
#79412=ORIENTED_EDGE('',*,*,#56640,.F.);
#79413=ORIENTED_EDGE('',*,*,#54490,.F.);
#79414=ORIENTED_EDGE('',*,*,#56639,.T.);
#79415=ORIENTED_EDGE('',*,*,#54478,.F.);
#79416=ORIENTED_EDGE('',*,*,#56641,.F.);
#79417=ORIENTED_EDGE('',*,*,#54744,.F.);
#79418=ORIENTED_EDGE('',*,*,#56640,.T.);
#79419=ORIENTED_EDGE('',*,*,#54747,.F.);
#79420=ORIENTED_EDGE('',*,*,#56642,.F.);
#79421=ORIENTED_EDGE('',*,*,#54469,.F.);
#79422=ORIENTED_EDGE('',*,*,#56641,.T.);
#79423=ORIENTED_EDGE('',*,*,#54496,.F.);
#79424=ORIENTED_EDGE('',*,*,#56643,.F.);
#79425=ORIENTED_EDGE('',*,*,#54745,.F.);
#79426=ORIENTED_EDGE('',*,*,#56642,.T.);
#79427=ORIENTED_EDGE('',*,*,#54746,.F.);
#79428=ORIENTED_EDGE('',*,*,#56643,.T.);
#79429=ORIENTED_EDGE('',*,*,#54474,.F.);
#79430=ORIENTED_EDGE('',*,*,#54470,.T.);
#79431=ORIENTED_EDGE('',*,*,#56644,.F.);
#79432=ORIENTED_EDGE('',*,*,#54786,.F.);
#79433=ORIENTED_EDGE('',*,*,#56645,.F.);
#79434=ORIENTED_EDGE('',*,*,#54426,.F.);
#79435=ORIENTED_EDGE('',*,*,#56645,.T.);
#79436=ORIENTED_EDGE('',*,*,#54785,.F.);
#79437=ORIENTED_EDGE('',*,*,#56646,.F.);
#79438=ORIENTED_EDGE('',*,*,#54435,.F.);
#79439=ORIENTED_EDGE('',*,*,#54425,.T.);
#79440=ORIENTED_EDGE('',*,*,#54429,.F.);
#79441=ORIENTED_EDGE('',*,*,#56647,.F.);
#79442=ORIENTED_EDGE('',*,*,#54787,.F.);
#79443=ORIENTED_EDGE('',*,*,#56644,.T.);
#79444=ORIENTED_EDGE('',*,*,#56646,.T.);
#79445=ORIENTED_EDGE('',*,*,#54784,.F.);
#79446=ORIENTED_EDGE('',*,*,#56648,.F.);
#79447=ORIENTED_EDGE('',*,*,#54420,.F.);
#79448=ORIENTED_EDGE('',*,*,#56647,.T.);
#79449=ORIENTED_EDGE('',*,*,#54433,.F.);
#79450=ORIENTED_EDGE('',*,*,#56649,.F.);
#79451=ORIENTED_EDGE('',*,*,#54776,.F.);
#79452=ORIENTED_EDGE('',*,*,#56648,.T.);
#79453=ORIENTED_EDGE('',*,*,#54783,.F.);
#79454=ORIENTED_EDGE('',*,*,#56650,.F.);
#79455=ORIENTED_EDGE('',*,*,#54437,.F.);
#79456=ORIENTED_EDGE('',*,*,#56649,.T.);
#79457=ORIENTED_EDGE('',*,*,#52096,.F.);
#79458=ORIENTED_EDGE('',*,*,#56651,.F.);
#79459=ORIENTED_EDGE('',*,*,#54777,.F.);
#79460=ORIENTED_EDGE('',*,*,#56650,.T.);
#79461=ORIENTED_EDGE('',*,*,#54782,.F.);
#79462=ORIENTED_EDGE('',*,*,#56652,.F.);
#79463=ORIENTED_EDGE('',*,*,#54412,.T.);
#79464=ORIENTED_EDGE('',*,*,#54416,.F.);
#79465=ORIENTED_EDGE('',*,*,#56651,.T.);
#79466=ORIENTED_EDGE('',*,*,#52095,.F.);
#79467=ORIENTED_EDGE('',*,*,#56653,.F.);
#79468=ORIENTED_EDGE('',*,*,#56312,.F.);
#79469=ORIENTED_EDGE('',*,*,#56652,.T.);
#79470=ORIENTED_EDGE('',*,*,#54781,.F.);
#79471=ORIENTED_EDGE('',*,*,#56654,.F.);
#79472=ORIENTED_EDGE('',*,*,#54413,.F.);
#79473=ORIENTED_EDGE('',*,*,#56653,.T.);
#79474=ORIENTED_EDGE('',*,*,#52094,.F.);
#79475=ORIENTED_EDGE('',*,*,#56655,.F.);
#79476=ORIENTED_EDGE('',*,*,#54761,.F.);
#79477=ORIENTED_EDGE('',*,*,#56654,.T.);
#79478=ORIENTED_EDGE('',*,*,#54780,.F.);
#79479=ORIENTED_EDGE('',*,*,#56656,.F.);
#79480=ORIENTED_EDGE('',*,*,#54431,.F.);
#79481=ORIENTED_EDGE('',*,*,#56655,.T.);
#79482=ORIENTED_EDGE('',*,*,#52093,.F.);
#79483=ORIENTED_EDGE('',*,*,#56657,.F.);
#79484=ORIENTED_EDGE('',*,*,#56314,.F.);
#79485=ORIENTED_EDGE('',*,*,#56656,.T.);
#79486=ORIENTED_EDGE('',*,*,#54779,.F.);
#79487=ORIENTED_EDGE('',*,*,#56658,.F.);
#79488=ORIENTED_EDGE('',*,*,#52570,.F.);
#79489=ORIENTED_EDGE('',*,*,#56657,.T.);
#79490=ORIENTED_EDGE('',*,*,#52092,.F.);
#79491=ORIENTED_EDGE('',*,*,#56659,.F.);
#79492=ORIENTED_EDGE('',*,*,#54767,.F.);
#79493=ORIENTED_EDGE('',*,*,#56658,.T.);
#79494=ORIENTED_EDGE('',*,*,#56313,.F.);
#79495=ORIENTED_EDGE('',*,*,#56660,.F.);
#79496=ORIENTED_EDGE('',*,*,#52571,.F.);
#79497=ORIENTED_EDGE('',*,*,#56659,.T.);
#79498=ORIENTED_EDGE('',*,*,#54462,.F.);
#79499=ORIENTED_EDGE('',*,*,#56661,.F.);
#79500=ORIENTED_EDGE('',*,*,#54768,.F.);
#79501=ORIENTED_EDGE('',*,*,#56660,.T.);
#79502=ORIENTED_EDGE('',*,*,#54763,.F.);
#79503=ORIENTED_EDGE('',*,*,#56662,.F.);
#79504=ORIENTED_EDGE('',*,*,#52572,.F.);
#79505=ORIENTED_EDGE('',*,*,#54457,.F.);
#79506=ORIENTED_EDGE('',*,*,#54453,.T.);
#79507=ORIENTED_EDGE('',*,*,#56663,.F.);
#79508=ORIENTED_EDGE('',*,*,#54769,.F.);
#79509=ORIENTED_EDGE('',*,*,#56661,.T.);
#79510=ORIENTED_EDGE('',*,*,#56662,.T.);
#79511=ORIENTED_EDGE('',*,*,#56315,.F.);
#79512=ORIENTED_EDGE('',*,*,#56664,.F.);
#79513=ORIENTED_EDGE('',*,*,#52573,.F.);
#79514=ORIENTED_EDGE('',*,*,#56663,.T.);
#79515=ORIENTED_EDGE('',*,*,#54452,.F.);
#79516=ORIENTED_EDGE('',*,*,#56665,.F.);
#79517=ORIENTED_EDGE('',*,*,#54770,.F.);
#79518=ORIENTED_EDGE('',*,*,#56664,.T.);
#79519=ORIENTED_EDGE('',*,*,#54765,.F.);
#79520=ORIENTED_EDGE('',*,*,#56666,.F.);
#79521=ORIENTED_EDGE('',*,*,#52574,.F.);
#79522=ORIENTED_EDGE('',*,*,#56665,.T.);
#79523=ORIENTED_EDGE('',*,*,#54464,.F.);
#79524=ORIENTED_EDGE('',*,*,#56667,.F.);
#79525=ORIENTED_EDGE('',*,*,#54771,.F.);
#79526=ORIENTED_EDGE('',*,*,#56666,.T.);
#79527=ORIENTED_EDGE('',*,*,#54764,.F.);
#79528=ORIENTED_EDGE('',*,*,#56668,.F.);
#79529=ORIENTED_EDGE('',*,*,#54460,.F.);
#79530=ORIENTED_EDGE('',*,*,#56667,.T.);
#79531=ORIENTED_EDGE('',*,*,#54448,.F.);
#79532=ORIENTED_EDGE('',*,*,#56669,.F.);
#79533=ORIENTED_EDGE('',*,*,#54772,.F.);
#79534=ORIENTED_EDGE('',*,*,#56668,.T.);
#79535=ORIENTED_EDGE('',*,*,#54775,.F.);
#79536=ORIENTED_EDGE('',*,*,#56670,.F.);
#79537=ORIENTED_EDGE('',*,*,#54439,.F.);
#79538=ORIENTED_EDGE('',*,*,#56669,.T.);
#79539=ORIENTED_EDGE('',*,*,#54466,.F.);
#79540=ORIENTED_EDGE('',*,*,#56671,.F.);
#79541=ORIENTED_EDGE('',*,*,#54773,.F.);
#79542=ORIENTED_EDGE('',*,*,#56670,.T.);
#79543=ORIENTED_EDGE('',*,*,#54774,.F.);
#79544=ORIENTED_EDGE('',*,*,#56671,.T.);
#79545=ORIENTED_EDGE('',*,*,#54444,.F.);
#79546=ORIENTED_EDGE('',*,*,#54440,.T.);
#79547=ORIENTED_EDGE('',*,*,#56672,.F.);
#79548=ORIENTED_EDGE('',*,*,#54814,.F.);
#79549=ORIENTED_EDGE('',*,*,#56673,.F.);
#79550=ORIENTED_EDGE('',*,*,#54396,.F.);
#79551=ORIENTED_EDGE('',*,*,#56673,.T.);
#79552=ORIENTED_EDGE('',*,*,#54813,.F.);
#79553=ORIENTED_EDGE('',*,*,#56674,.F.);
#79554=ORIENTED_EDGE('',*,*,#54405,.F.);
#79555=ORIENTED_EDGE('',*,*,#54395,.T.);
#79556=ORIENTED_EDGE('',*,*,#54399,.F.);
#79557=ORIENTED_EDGE('',*,*,#56675,.F.);
#79558=ORIENTED_EDGE('',*,*,#54815,.F.);
#79559=ORIENTED_EDGE('',*,*,#56672,.T.);
#79560=ORIENTED_EDGE('',*,*,#56674,.T.);
#79561=ORIENTED_EDGE('',*,*,#54812,.F.);
#79562=ORIENTED_EDGE('',*,*,#56676,.F.);
#79563=ORIENTED_EDGE('',*,*,#54390,.F.);
#79564=ORIENTED_EDGE('',*,*,#56675,.T.);
#79565=ORIENTED_EDGE('',*,*,#54403,.F.);
#79566=ORIENTED_EDGE('',*,*,#56677,.F.);
#79567=ORIENTED_EDGE('',*,*,#54804,.F.);
#79568=ORIENTED_EDGE('',*,*,#56676,.T.);
#79569=ORIENTED_EDGE('',*,*,#54811,.F.);
#79570=ORIENTED_EDGE('',*,*,#56678,.F.);
#79571=ORIENTED_EDGE('',*,*,#54407,.F.);
#79572=ORIENTED_EDGE('',*,*,#56677,.T.);
#79573=ORIENTED_EDGE('',*,*,#52102,.F.);
#79574=ORIENTED_EDGE('',*,*,#56679,.F.);
#79575=ORIENTED_EDGE('',*,*,#54805,.F.);
#79576=ORIENTED_EDGE('',*,*,#56678,.T.);
#79577=ORIENTED_EDGE('',*,*,#54810,.F.);
#79578=ORIENTED_EDGE('',*,*,#56680,.F.);
#79579=ORIENTED_EDGE('',*,*,#54382,.T.);
#79580=ORIENTED_EDGE('',*,*,#54386,.F.);
#79581=ORIENTED_EDGE('',*,*,#56679,.T.);
#79582=ORIENTED_EDGE('',*,*,#52101,.F.);
#79583=ORIENTED_EDGE('',*,*,#56681,.F.);
#79584=ORIENTED_EDGE('',*,*,#56316,.F.);
#79585=ORIENTED_EDGE('',*,*,#56680,.T.);
#79586=ORIENTED_EDGE('',*,*,#54809,.F.);
#79587=ORIENTED_EDGE('',*,*,#56682,.F.);
#79588=ORIENTED_EDGE('',*,*,#54383,.F.);
#79589=ORIENTED_EDGE('',*,*,#56681,.T.);
#79590=ORIENTED_EDGE('',*,*,#52100,.F.);
#79591=ORIENTED_EDGE('',*,*,#56683,.F.);
#79592=ORIENTED_EDGE('',*,*,#54789,.F.);
#79593=ORIENTED_EDGE('',*,*,#56682,.T.);
#79594=ORIENTED_EDGE('',*,*,#54808,.F.);
#79595=ORIENTED_EDGE('',*,*,#56684,.F.);
#79596=ORIENTED_EDGE('',*,*,#54401,.F.);
#79597=ORIENTED_EDGE('',*,*,#56683,.T.);
#79598=ORIENTED_EDGE('',*,*,#52099,.F.);
#79599=ORIENTED_EDGE('',*,*,#56685,.F.);
#79600=ORIENTED_EDGE('',*,*,#56318,.F.);
#79601=ORIENTED_EDGE('',*,*,#56684,.T.);
#79602=ORIENTED_EDGE('',*,*,#54807,.F.);
#79603=ORIENTED_EDGE('',*,*,#56686,.F.);
#79604=ORIENTED_EDGE('',*,*,#52564,.F.);
#79605=ORIENTED_EDGE('',*,*,#56685,.T.);
#79606=ORIENTED_EDGE('',*,*,#52098,.F.);
#79607=ORIENTED_EDGE('',*,*,#56687,.F.);
#79608=ORIENTED_EDGE('',*,*,#54795,.F.);
#79609=ORIENTED_EDGE('',*,*,#56686,.T.);
#79610=ORIENTED_EDGE('',*,*,#56317,.F.);
#79611=ORIENTED_EDGE('',*,*,#56688,.F.);
#79612=ORIENTED_EDGE('',*,*,#52565,.F.);
#79613=ORIENTED_EDGE('',*,*,#56687,.T.);
#79614=ORIENTED_EDGE('',*,*,#54432,.F.);
#79615=ORIENTED_EDGE('',*,*,#56689,.F.);
#79616=ORIENTED_EDGE('',*,*,#54796,.F.);
#79617=ORIENTED_EDGE('',*,*,#56688,.T.);
#79618=ORIENTED_EDGE('',*,*,#54791,.F.);
#79619=ORIENTED_EDGE('',*,*,#56690,.F.);
#79620=ORIENTED_EDGE('',*,*,#52566,.F.);
#79621=ORIENTED_EDGE('',*,*,#54427,.F.);
#79622=ORIENTED_EDGE('',*,*,#54423,.T.);
#79623=ORIENTED_EDGE('',*,*,#56691,.F.);
#79624=ORIENTED_EDGE('',*,*,#54797,.F.);
#79625=ORIENTED_EDGE('',*,*,#56689,.T.);
#79626=ORIENTED_EDGE('',*,*,#56690,.T.);
#79627=ORIENTED_EDGE('',*,*,#56319,.F.);
#79628=ORIENTED_EDGE('',*,*,#56692,.F.);
#79629=ORIENTED_EDGE('',*,*,#52567,.F.);
#79630=ORIENTED_EDGE('',*,*,#56691,.T.);
#79631=ORIENTED_EDGE('',*,*,#54422,.F.);
#79632=ORIENTED_EDGE('',*,*,#56693,.F.);
#79633=ORIENTED_EDGE('',*,*,#54798,.F.);
#79634=ORIENTED_EDGE('',*,*,#56692,.T.);
#79635=ORIENTED_EDGE('',*,*,#54793,.F.);
#79636=ORIENTED_EDGE('',*,*,#56694,.F.);
#79637=ORIENTED_EDGE('',*,*,#52568,.F.);
#79638=ORIENTED_EDGE('',*,*,#56693,.T.);
#79639=ORIENTED_EDGE('',*,*,#54434,.F.);
#79640=ORIENTED_EDGE('',*,*,#56695,.F.);
#79641=ORIENTED_EDGE('',*,*,#54799,.F.);
#79642=ORIENTED_EDGE('',*,*,#56694,.T.);
#79643=ORIENTED_EDGE('',*,*,#54792,.F.);
#79644=ORIENTED_EDGE('',*,*,#56696,.F.);
#79645=ORIENTED_EDGE('',*,*,#54430,.F.);
#79646=ORIENTED_EDGE('',*,*,#56695,.T.);
#79647=ORIENTED_EDGE('',*,*,#54418,.F.);
#79648=ORIENTED_EDGE('',*,*,#56697,.F.);
#79649=ORIENTED_EDGE('',*,*,#54800,.F.);
#79650=ORIENTED_EDGE('',*,*,#56696,.T.);
#79651=ORIENTED_EDGE('',*,*,#54803,.F.);
#79652=ORIENTED_EDGE('',*,*,#56698,.F.);
#79653=ORIENTED_EDGE('',*,*,#54409,.F.);
#79654=ORIENTED_EDGE('',*,*,#56697,.T.);
#79655=ORIENTED_EDGE('',*,*,#54436,.F.);
#79656=ORIENTED_EDGE('',*,*,#56699,.F.);
#79657=ORIENTED_EDGE('',*,*,#54801,.F.);
#79658=ORIENTED_EDGE('',*,*,#56698,.T.);
#79659=ORIENTED_EDGE('',*,*,#54802,.F.);
#79660=ORIENTED_EDGE('',*,*,#56699,.T.);
#79661=ORIENTED_EDGE('',*,*,#54414,.F.);
#79662=ORIENTED_EDGE('',*,*,#54410,.T.);
#79663=ORIENTED_EDGE('',*,*,#56700,.F.);
#79664=ORIENTED_EDGE('',*,*,#54842,.F.);
#79665=ORIENTED_EDGE('',*,*,#56701,.F.);
#79666=ORIENTED_EDGE('',*,*,#54366,.F.);
#79667=ORIENTED_EDGE('',*,*,#56701,.T.);
#79668=ORIENTED_EDGE('',*,*,#54841,.F.);
#79669=ORIENTED_EDGE('',*,*,#56702,.F.);
#79670=ORIENTED_EDGE('',*,*,#54375,.F.);
#79671=ORIENTED_EDGE('',*,*,#54365,.T.);
#79672=ORIENTED_EDGE('',*,*,#54369,.F.);
#79673=ORIENTED_EDGE('',*,*,#56703,.F.);
#79674=ORIENTED_EDGE('',*,*,#54843,.F.);
#79675=ORIENTED_EDGE('',*,*,#56700,.T.);
#79676=ORIENTED_EDGE('',*,*,#56702,.T.);
#79677=ORIENTED_EDGE('',*,*,#54840,.F.);
#79678=ORIENTED_EDGE('',*,*,#56704,.F.);
#79679=ORIENTED_EDGE('',*,*,#54360,.F.);
#79680=ORIENTED_EDGE('',*,*,#56703,.T.);
#79681=ORIENTED_EDGE('',*,*,#54373,.F.);
#79682=ORIENTED_EDGE('',*,*,#56705,.F.);
#79683=ORIENTED_EDGE('',*,*,#54832,.F.);
#79684=ORIENTED_EDGE('',*,*,#56704,.T.);
#79685=ORIENTED_EDGE('',*,*,#54839,.F.);
#79686=ORIENTED_EDGE('',*,*,#56706,.F.);
#79687=ORIENTED_EDGE('',*,*,#54377,.F.);
#79688=ORIENTED_EDGE('',*,*,#56705,.T.);
#79689=ORIENTED_EDGE('',*,*,#52108,.F.);
#79690=ORIENTED_EDGE('',*,*,#56707,.F.);
#79691=ORIENTED_EDGE('',*,*,#54833,.F.);
#79692=ORIENTED_EDGE('',*,*,#56706,.T.);
#79693=ORIENTED_EDGE('',*,*,#54838,.F.);
#79694=ORIENTED_EDGE('',*,*,#56708,.F.);
#79695=ORIENTED_EDGE('',*,*,#54352,.T.);
#79696=ORIENTED_EDGE('',*,*,#54356,.F.);
#79697=ORIENTED_EDGE('',*,*,#56707,.T.);
#79698=ORIENTED_EDGE('',*,*,#52107,.F.);
#79699=ORIENTED_EDGE('',*,*,#56709,.F.);
#79700=ORIENTED_EDGE('',*,*,#56320,.F.);
#79701=ORIENTED_EDGE('',*,*,#56708,.T.);
#79702=ORIENTED_EDGE('',*,*,#54837,.F.);
#79703=ORIENTED_EDGE('',*,*,#56710,.F.);
#79704=ORIENTED_EDGE('',*,*,#54353,.F.);
#79705=ORIENTED_EDGE('',*,*,#56709,.T.);
#79706=ORIENTED_EDGE('',*,*,#52106,.F.);
#79707=ORIENTED_EDGE('',*,*,#56711,.F.);
#79708=ORIENTED_EDGE('',*,*,#54817,.F.);
#79709=ORIENTED_EDGE('',*,*,#56710,.T.);
#79710=ORIENTED_EDGE('',*,*,#54836,.F.);
#79711=ORIENTED_EDGE('',*,*,#56712,.F.);
#79712=ORIENTED_EDGE('',*,*,#54371,.F.);
#79713=ORIENTED_EDGE('',*,*,#56711,.T.);
#79714=ORIENTED_EDGE('',*,*,#52105,.F.);
#79715=ORIENTED_EDGE('',*,*,#56713,.F.);
#79716=ORIENTED_EDGE('',*,*,#56322,.F.);
#79717=ORIENTED_EDGE('',*,*,#56712,.T.);
#79718=ORIENTED_EDGE('',*,*,#54835,.F.);
#79719=ORIENTED_EDGE('',*,*,#56714,.F.);
#79720=ORIENTED_EDGE('',*,*,#52558,.F.);
#79721=ORIENTED_EDGE('',*,*,#56713,.T.);
#79722=ORIENTED_EDGE('',*,*,#52104,.F.);
#79723=ORIENTED_EDGE('',*,*,#56715,.F.);
#79724=ORIENTED_EDGE('',*,*,#54823,.F.);
#79725=ORIENTED_EDGE('',*,*,#56714,.T.);
#79726=ORIENTED_EDGE('',*,*,#56321,.F.);
#79727=ORIENTED_EDGE('',*,*,#56716,.F.);
#79728=ORIENTED_EDGE('',*,*,#52559,.F.);
#79729=ORIENTED_EDGE('',*,*,#56715,.T.);
#79730=ORIENTED_EDGE('',*,*,#54402,.F.);
#79731=ORIENTED_EDGE('',*,*,#56717,.F.);
#79732=ORIENTED_EDGE('',*,*,#54824,.F.);
#79733=ORIENTED_EDGE('',*,*,#56716,.T.);
#79734=ORIENTED_EDGE('',*,*,#54819,.F.);
#79735=ORIENTED_EDGE('',*,*,#56718,.F.);
#79736=ORIENTED_EDGE('',*,*,#52560,.F.);
#79737=ORIENTED_EDGE('',*,*,#54397,.F.);
#79738=ORIENTED_EDGE('',*,*,#54393,.T.);
#79739=ORIENTED_EDGE('',*,*,#56719,.F.);
#79740=ORIENTED_EDGE('',*,*,#54825,.F.);
#79741=ORIENTED_EDGE('',*,*,#56717,.T.);
#79742=ORIENTED_EDGE('',*,*,#56718,.T.);
#79743=ORIENTED_EDGE('',*,*,#56323,.F.);
#79744=ORIENTED_EDGE('',*,*,#56720,.F.);
#79745=ORIENTED_EDGE('',*,*,#52561,.F.);
#79746=ORIENTED_EDGE('',*,*,#56719,.T.);
#79747=ORIENTED_EDGE('',*,*,#54392,.F.);
#79748=ORIENTED_EDGE('',*,*,#56721,.F.);
#79749=ORIENTED_EDGE('',*,*,#54826,.F.);
#79750=ORIENTED_EDGE('',*,*,#56720,.T.);
#79751=ORIENTED_EDGE('',*,*,#54821,.F.);
#79752=ORIENTED_EDGE('',*,*,#56722,.F.);
#79753=ORIENTED_EDGE('',*,*,#52562,.F.);
#79754=ORIENTED_EDGE('',*,*,#56721,.T.);
#79755=ORIENTED_EDGE('',*,*,#54404,.F.);
#79756=ORIENTED_EDGE('',*,*,#56723,.F.);
#79757=ORIENTED_EDGE('',*,*,#54827,.F.);
#79758=ORIENTED_EDGE('',*,*,#56722,.T.);
#79759=ORIENTED_EDGE('',*,*,#54820,.F.);
#79760=ORIENTED_EDGE('',*,*,#56724,.F.);
#79761=ORIENTED_EDGE('',*,*,#54400,.F.);
#79762=ORIENTED_EDGE('',*,*,#56723,.T.);
#79763=ORIENTED_EDGE('',*,*,#54388,.F.);
#79764=ORIENTED_EDGE('',*,*,#56725,.F.);
#79765=ORIENTED_EDGE('',*,*,#54828,.F.);
#79766=ORIENTED_EDGE('',*,*,#56724,.T.);
#79767=ORIENTED_EDGE('',*,*,#54831,.F.);
#79768=ORIENTED_EDGE('',*,*,#56726,.F.);
#79769=ORIENTED_EDGE('',*,*,#54379,.F.);
#79770=ORIENTED_EDGE('',*,*,#56725,.T.);
#79771=ORIENTED_EDGE('',*,*,#54406,.F.);
#79772=ORIENTED_EDGE('',*,*,#56727,.F.);
#79773=ORIENTED_EDGE('',*,*,#54829,.F.);
#79774=ORIENTED_EDGE('',*,*,#56726,.T.);
#79775=ORIENTED_EDGE('',*,*,#54830,.F.);
#79776=ORIENTED_EDGE('',*,*,#56727,.T.);
#79777=ORIENTED_EDGE('',*,*,#54384,.F.);
#79778=ORIENTED_EDGE('',*,*,#54380,.T.);
#79779=ORIENTED_EDGE('',*,*,#56728,.F.);
#79780=ORIENTED_EDGE('',*,*,#54870,.F.);
#79781=ORIENTED_EDGE('',*,*,#56729,.F.);
#79782=ORIENTED_EDGE('',*,*,#54336,.F.);
#79783=ORIENTED_EDGE('',*,*,#56729,.T.);
#79784=ORIENTED_EDGE('',*,*,#54869,.F.);
#79785=ORIENTED_EDGE('',*,*,#56730,.F.);
#79786=ORIENTED_EDGE('',*,*,#54345,.F.);
#79787=ORIENTED_EDGE('',*,*,#54335,.T.);
#79788=ORIENTED_EDGE('',*,*,#54339,.F.);
#79789=ORIENTED_EDGE('',*,*,#56731,.F.);
#79790=ORIENTED_EDGE('',*,*,#54871,.F.);
#79791=ORIENTED_EDGE('',*,*,#56728,.T.);
#79792=ORIENTED_EDGE('',*,*,#56730,.T.);
#79793=ORIENTED_EDGE('',*,*,#54868,.F.);
#79794=ORIENTED_EDGE('',*,*,#56732,.F.);
#79795=ORIENTED_EDGE('',*,*,#54330,.F.);
#79796=ORIENTED_EDGE('',*,*,#56731,.T.);
#79797=ORIENTED_EDGE('',*,*,#54343,.F.);
#79798=ORIENTED_EDGE('',*,*,#56733,.F.);
#79799=ORIENTED_EDGE('',*,*,#54860,.F.);
#79800=ORIENTED_EDGE('',*,*,#56732,.T.);
#79801=ORIENTED_EDGE('',*,*,#54867,.F.);
#79802=ORIENTED_EDGE('',*,*,#56734,.F.);
#79803=ORIENTED_EDGE('',*,*,#54347,.F.);
#79804=ORIENTED_EDGE('',*,*,#56733,.T.);
#79805=ORIENTED_EDGE('',*,*,#52114,.F.);
#79806=ORIENTED_EDGE('',*,*,#56735,.F.);
#79807=ORIENTED_EDGE('',*,*,#54861,.F.);
#79808=ORIENTED_EDGE('',*,*,#56734,.T.);
#79809=ORIENTED_EDGE('',*,*,#54866,.F.);
#79810=ORIENTED_EDGE('',*,*,#56736,.F.);
#79811=ORIENTED_EDGE('',*,*,#54322,.T.);
#79812=ORIENTED_EDGE('',*,*,#54326,.F.);
#79813=ORIENTED_EDGE('',*,*,#56735,.T.);
#79814=ORIENTED_EDGE('',*,*,#52113,.F.);
#79815=ORIENTED_EDGE('',*,*,#56737,.F.);
#79816=ORIENTED_EDGE('',*,*,#56324,.F.);
#79817=ORIENTED_EDGE('',*,*,#56736,.T.);
#79818=ORIENTED_EDGE('',*,*,#54865,.F.);
#79819=ORIENTED_EDGE('',*,*,#56738,.F.);
#79820=ORIENTED_EDGE('',*,*,#54323,.F.);
#79821=ORIENTED_EDGE('',*,*,#56737,.T.);
#79822=ORIENTED_EDGE('',*,*,#52112,.F.);
#79823=ORIENTED_EDGE('',*,*,#56739,.F.);
#79824=ORIENTED_EDGE('',*,*,#54845,.F.);
#79825=ORIENTED_EDGE('',*,*,#56738,.T.);
#79826=ORIENTED_EDGE('',*,*,#54864,.F.);
#79827=ORIENTED_EDGE('',*,*,#56740,.F.);
#79828=ORIENTED_EDGE('',*,*,#54341,.F.);
#79829=ORIENTED_EDGE('',*,*,#56739,.T.);
#79830=ORIENTED_EDGE('',*,*,#52111,.F.);
#79831=ORIENTED_EDGE('',*,*,#56741,.F.);
#79832=ORIENTED_EDGE('',*,*,#56326,.F.);
#79833=ORIENTED_EDGE('',*,*,#56740,.T.);
#79834=ORIENTED_EDGE('',*,*,#54863,.F.);
#79835=ORIENTED_EDGE('',*,*,#56742,.F.);
#79836=ORIENTED_EDGE('',*,*,#52552,.F.);
#79837=ORIENTED_EDGE('',*,*,#56741,.T.);
#79838=ORIENTED_EDGE('',*,*,#52110,.F.);
#79839=ORIENTED_EDGE('',*,*,#56743,.F.);
#79840=ORIENTED_EDGE('',*,*,#54851,.F.);
#79841=ORIENTED_EDGE('',*,*,#56742,.T.);
#79842=ORIENTED_EDGE('',*,*,#56325,.F.);
#79843=ORIENTED_EDGE('',*,*,#56744,.F.);
#79844=ORIENTED_EDGE('',*,*,#52553,.F.);
#79845=ORIENTED_EDGE('',*,*,#56743,.T.);
#79846=ORIENTED_EDGE('',*,*,#54372,.F.);
#79847=ORIENTED_EDGE('',*,*,#56745,.F.);
#79848=ORIENTED_EDGE('',*,*,#54852,.F.);
#79849=ORIENTED_EDGE('',*,*,#56744,.T.);
#79850=ORIENTED_EDGE('',*,*,#54847,.F.);
#79851=ORIENTED_EDGE('',*,*,#56746,.F.);
#79852=ORIENTED_EDGE('',*,*,#52554,.F.);
#79853=ORIENTED_EDGE('',*,*,#54367,.F.);
#79854=ORIENTED_EDGE('',*,*,#54363,.T.);
#79855=ORIENTED_EDGE('',*,*,#56747,.F.);
#79856=ORIENTED_EDGE('',*,*,#54853,.F.);
#79857=ORIENTED_EDGE('',*,*,#56745,.T.);
#79858=ORIENTED_EDGE('',*,*,#56746,.T.);
#79859=ORIENTED_EDGE('',*,*,#56327,.F.);
#79860=ORIENTED_EDGE('',*,*,#56748,.F.);
#79861=ORIENTED_EDGE('',*,*,#52555,.F.);
#79862=ORIENTED_EDGE('',*,*,#56747,.T.);
#79863=ORIENTED_EDGE('',*,*,#54362,.F.);
#79864=ORIENTED_EDGE('',*,*,#56749,.F.);
#79865=ORIENTED_EDGE('',*,*,#54854,.F.);
#79866=ORIENTED_EDGE('',*,*,#56748,.T.);
#79867=ORIENTED_EDGE('',*,*,#54849,.F.);
#79868=ORIENTED_EDGE('',*,*,#56750,.F.);
#79869=ORIENTED_EDGE('',*,*,#52556,.F.);
#79870=ORIENTED_EDGE('',*,*,#56749,.T.);
#79871=ORIENTED_EDGE('',*,*,#54374,.F.);
#79872=ORIENTED_EDGE('',*,*,#56751,.F.);
#79873=ORIENTED_EDGE('',*,*,#54855,.F.);
#79874=ORIENTED_EDGE('',*,*,#56750,.T.);
#79875=ORIENTED_EDGE('',*,*,#54848,.F.);
#79876=ORIENTED_EDGE('',*,*,#56752,.F.);
#79877=ORIENTED_EDGE('',*,*,#54370,.F.);
#79878=ORIENTED_EDGE('',*,*,#56751,.T.);
#79879=ORIENTED_EDGE('',*,*,#54358,.F.);
#79880=ORIENTED_EDGE('',*,*,#56753,.F.);
#79881=ORIENTED_EDGE('',*,*,#54856,.F.);
#79882=ORIENTED_EDGE('',*,*,#56752,.T.);
#79883=ORIENTED_EDGE('',*,*,#54859,.F.);
#79884=ORIENTED_EDGE('',*,*,#56754,.F.);
#79885=ORIENTED_EDGE('',*,*,#54349,.F.);
#79886=ORIENTED_EDGE('',*,*,#56753,.T.);
#79887=ORIENTED_EDGE('',*,*,#54376,.F.);
#79888=ORIENTED_EDGE('',*,*,#56755,.F.);
#79889=ORIENTED_EDGE('',*,*,#54857,.F.);
#79890=ORIENTED_EDGE('',*,*,#56754,.T.);
#79891=ORIENTED_EDGE('',*,*,#54858,.F.);
#79892=ORIENTED_EDGE('',*,*,#56755,.T.);
#79893=ORIENTED_EDGE('',*,*,#54354,.F.);
#79894=ORIENTED_EDGE('',*,*,#54350,.T.);
#79895=ORIENTED_EDGE('',*,*,#56756,.F.);
#79896=ORIENTED_EDGE('',*,*,#54898,.F.);
#79897=ORIENTED_EDGE('',*,*,#56757,.F.);
#79898=ORIENTED_EDGE('',*,*,#54306,.F.);
#79899=ORIENTED_EDGE('',*,*,#56757,.T.);
#79900=ORIENTED_EDGE('',*,*,#54897,.F.);
#79901=ORIENTED_EDGE('',*,*,#56758,.F.);
#79902=ORIENTED_EDGE('',*,*,#54315,.F.);
#79903=ORIENTED_EDGE('',*,*,#54305,.T.);
#79904=ORIENTED_EDGE('',*,*,#54309,.F.);
#79905=ORIENTED_EDGE('',*,*,#56759,.F.);
#79906=ORIENTED_EDGE('',*,*,#54899,.F.);
#79907=ORIENTED_EDGE('',*,*,#56756,.T.);
#79908=ORIENTED_EDGE('',*,*,#56758,.T.);
#79909=ORIENTED_EDGE('',*,*,#54896,.F.);
#79910=ORIENTED_EDGE('',*,*,#56760,.F.);
#79911=ORIENTED_EDGE('',*,*,#54300,.F.);
#79912=ORIENTED_EDGE('',*,*,#56759,.T.);
#79913=ORIENTED_EDGE('',*,*,#54313,.F.);
#79914=ORIENTED_EDGE('',*,*,#56761,.F.);
#79915=ORIENTED_EDGE('',*,*,#54888,.F.);
#79916=ORIENTED_EDGE('',*,*,#56760,.T.);
#79917=ORIENTED_EDGE('',*,*,#54895,.F.);
#79918=ORIENTED_EDGE('',*,*,#56762,.F.);
#79919=ORIENTED_EDGE('',*,*,#54317,.F.);
#79920=ORIENTED_EDGE('',*,*,#56761,.T.);
#79921=ORIENTED_EDGE('',*,*,#52120,.F.);
#79922=ORIENTED_EDGE('',*,*,#56763,.F.);
#79923=ORIENTED_EDGE('',*,*,#54889,.F.);
#79924=ORIENTED_EDGE('',*,*,#56762,.T.);
#79925=ORIENTED_EDGE('',*,*,#54894,.F.);
#79926=ORIENTED_EDGE('',*,*,#56764,.F.);
#79927=ORIENTED_EDGE('',*,*,#54292,.T.);
#79928=ORIENTED_EDGE('',*,*,#54296,.F.);
#79929=ORIENTED_EDGE('',*,*,#56763,.T.);
#79930=ORIENTED_EDGE('',*,*,#52119,.F.);
#79931=ORIENTED_EDGE('',*,*,#56765,.F.);
#79932=ORIENTED_EDGE('',*,*,#56328,.F.);
#79933=ORIENTED_EDGE('',*,*,#56764,.T.);
#79934=ORIENTED_EDGE('',*,*,#54893,.F.);
#79935=ORIENTED_EDGE('',*,*,#56766,.F.);
#79936=ORIENTED_EDGE('',*,*,#54293,.F.);
#79937=ORIENTED_EDGE('',*,*,#56765,.T.);
#79938=ORIENTED_EDGE('',*,*,#52118,.F.);
#79939=ORIENTED_EDGE('',*,*,#56767,.F.);
#79940=ORIENTED_EDGE('',*,*,#54873,.F.);
#79941=ORIENTED_EDGE('',*,*,#56766,.T.);
#79942=ORIENTED_EDGE('',*,*,#54892,.F.);
#79943=ORIENTED_EDGE('',*,*,#56768,.F.);
#79944=ORIENTED_EDGE('',*,*,#54311,.F.);
#79945=ORIENTED_EDGE('',*,*,#56767,.T.);
#79946=ORIENTED_EDGE('',*,*,#52117,.F.);
#79947=ORIENTED_EDGE('',*,*,#56769,.F.);
#79948=ORIENTED_EDGE('',*,*,#56330,.F.);
#79949=ORIENTED_EDGE('',*,*,#56768,.T.);
#79950=ORIENTED_EDGE('',*,*,#54891,.F.);
#79951=ORIENTED_EDGE('',*,*,#56770,.F.);
#79952=ORIENTED_EDGE('',*,*,#52546,.F.);
#79953=ORIENTED_EDGE('',*,*,#56769,.T.);
#79954=ORIENTED_EDGE('',*,*,#52116,.F.);
#79955=ORIENTED_EDGE('',*,*,#56771,.F.);
#79956=ORIENTED_EDGE('',*,*,#54879,.F.);
#79957=ORIENTED_EDGE('',*,*,#56770,.T.);
#79958=ORIENTED_EDGE('',*,*,#56329,.F.);
#79959=ORIENTED_EDGE('',*,*,#56772,.F.);
#79960=ORIENTED_EDGE('',*,*,#52547,.F.);
#79961=ORIENTED_EDGE('',*,*,#56771,.T.);
#79962=ORIENTED_EDGE('',*,*,#54342,.F.);
#79963=ORIENTED_EDGE('',*,*,#56773,.F.);
#79964=ORIENTED_EDGE('',*,*,#54880,.F.);
#79965=ORIENTED_EDGE('',*,*,#56772,.T.);
#79966=ORIENTED_EDGE('',*,*,#54875,.F.);
#79967=ORIENTED_EDGE('',*,*,#56774,.F.);
#79968=ORIENTED_EDGE('',*,*,#52548,.F.);
#79969=ORIENTED_EDGE('',*,*,#54337,.F.);
#79970=ORIENTED_EDGE('',*,*,#54333,.T.);
#79971=ORIENTED_EDGE('',*,*,#56775,.F.);
#79972=ORIENTED_EDGE('',*,*,#54881,.F.);
#79973=ORIENTED_EDGE('',*,*,#56773,.T.);
#79974=ORIENTED_EDGE('',*,*,#56774,.T.);
#79975=ORIENTED_EDGE('',*,*,#56331,.F.);
#79976=ORIENTED_EDGE('',*,*,#56776,.F.);
#79977=ORIENTED_EDGE('',*,*,#52549,.F.);
#79978=ORIENTED_EDGE('',*,*,#56775,.T.);
#79979=ORIENTED_EDGE('',*,*,#54332,.F.);
#79980=ORIENTED_EDGE('',*,*,#56777,.F.);
#79981=ORIENTED_EDGE('',*,*,#54882,.F.);
#79982=ORIENTED_EDGE('',*,*,#56776,.T.);
#79983=ORIENTED_EDGE('',*,*,#54877,.F.);
#79984=ORIENTED_EDGE('',*,*,#56778,.F.);
#79985=ORIENTED_EDGE('',*,*,#52550,.F.);
#79986=ORIENTED_EDGE('',*,*,#56777,.T.);
#79987=ORIENTED_EDGE('',*,*,#54344,.F.);
#79988=ORIENTED_EDGE('',*,*,#56779,.F.);
#79989=ORIENTED_EDGE('',*,*,#54883,.F.);
#79990=ORIENTED_EDGE('',*,*,#56778,.T.);
#79991=ORIENTED_EDGE('',*,*,#54876,.F.);
#79992=ORIENTED_EDGE('',*,*,#56780,.F.);
#79993=ORIENTED_EDGE('',*,*,#54340,.F.);
#79994=ORIENTED_EDGE('',*,*,#56779,.T.);
#79995=ORIENTED_EDGE('',*,*,#54328,.F.);
#79996=ORIENTED_EDGE('',*,*,#56781,.F.);
#79997=ORIENTED_EDGE('',*,*,#54884,.F.);
#79998=ORIENTED_EDGE('',*,*,#56780,.T.);
#79999=ORIENTED_EDGE('',*,*,#54887,.F.);
#80000=ORIENTED_EDGE('',*,*,#56782,.F.);
#80001=ORIENTED_EDGE('',*,*,#54319,.F.);
#80002=ORIENTED_EDGE('',*,*,#56781,.T.);
#80003=ORIENTED_EDGE('',*,*,#54346,.F.);
#80004=ORIENTED_EDGE('',*,*,#56783,.F.);
#80005=ORIENTED_EDGE('',*,*,#54885,.F.);
#80006=ORIENTED_EDGE('',*,*,#56782,.T.);
#80007=ORIENTED_EDGE('',*,*,#54886,.F.);
#80008=ORIENTED_EDGE('',*,*,#56783,.T.);
#80009=ORIENTED_EDGE('',*,*,#54324,.F.);
#80010=ORIENTED_EDGE('',*,*,#54320,.T.);
#80011=ORIENTED_EDGE('',*,*,#56784,.F.);
#80012=ORIENTED_EDGE('',*,*,#54926,.F.);
#80013=ORIENTED_EDGE('',*,*,#56785,.F.);
#80014=ORIENTED_EDGE('',*,*,#54276,.F.);
#80015=ORIENTED_EDGE('',*,*,#56785,.T.);
#80016=ORIENTED_EDGE('',*,*,#54925,.F.);
#80017=ORIENTED_EDGE('',*,*,#56786,.F.);
#80018=ORIENTED_EDGE('',*,*,#54285,.F.);
#80019=ORIENTED_EDGE('',*,*,#54275,.T.);
#80020=ORIENTED_EDGE('',*,*,#54279,.F.);
#80021=ORIENTED_EDGE('',*,*,#56787,.F.);
#80022=ORIENTED_EDGE('',*,*,#54927,.F.);
#80023=ORIENTED_EDGE('',*,*,#56784,.T.);
#80024=ORIENTED_EDGE('',*,*,#56786,.T.);
#80025=ORIENTED_EDGE('',*,*,#54924,.F.);
#80026=ORIENTED_EDGE('',*,*,#56788,.F.);
#80027=ORIENTED_EDGE('',*,*,#54270,.F.);
#80028=ORIENTED_EDGE('',*,*,#56787,.T.);
#80029=ORIENTED_EDGE('',*,*,#54283,.F.);
#80030=ORIENTED_EDGE('',*,*,#56789,.F.);
#80031=ORIENTED_EDGE('',*,*,#54916,.F.);
#80032=ORIENTED_EDGE('',*,*,#56788,.T.);
#80033=ORIENTED_EDGE('',*,*,#54923,.F.);
#80034=ORIENTED_EDGE('',*,*,#56790,.F.);
#80035=ORIENTED_EDGE('',*,*,#54287,.F.);
#80036=ORIENTED_EDGE('',*,*,#56789,.T.);
#80037=ORIENTED_EDGE('',*,*,#52126,.F.);
#80038=ORIENTED_EDGE('',*,*,#56791,.F.);
#80039=ORIENTED_EDGE('',*,*,#54917,.F.);
#80040=ORIENTED_EDGE('',*,*,#56790,.T.);
#80041=ORIENTED_EDGE('',*,*,#54922,.F.);
#80042=ORIENTED_EDGE('',*,*,#56792,.F.);
#80043=ORIENTED_EDGE('',*,*,#54262,.T.);
#80044=ORIENTED_EDGE('',*,*,#54266,.F.);
#80045=ORIENTED_EDGE('',*,*,#56791,.T.);
#80046=ORIENTED_EDGE('',*,*,#52125,.F.);
#80047=ORIENTED_EDGE('',*,*,#56793,.F.);
#80048=ORIENTED_EDGE('',*,*,#56332,.F.);
#80049=ORIENTED_EDGE('',*,*,#56792,.T.);
#80050=ORIENTED_EDGE('',*,*,#54921,.F.);
#80051=ORIENTED_EDGE('',*,*,#56794,.F.);
#80052=ORIENTED_EDGE('',*,*,#54263,.F.);
#80053=ORIENTED_EDGE('',*,*,#56793,.T.);
#80054=ORIENTED_EDGE('',*,*,#52124,.F.);
#80055=ORIENTED_EDGE('',*,*,#56795,.F.);
#80056=ORIENTED_EDGE('',*,*,#54901,.F.);
#80057=ORIENTED_EDGE('',*,*,#56794,.T.);
#80058=ORIENTED_EDGE('',*,*,#54920,.F.);
#80059=ORIENTED_EDGE('',*,*,#56796,.F.);
#80060=ORIENTED_EDGE('',*,*,#54281,.F.);
#80061=ORIENTED_EDGE('',*,*,#56795,.T.);
#80062=ORIENTED_EDGE('',*,*,#52123,.F.);
#80063=ORIENTED_EDGE('',*,*,#56797,.F.);
#80064=ORIENTED_EDGE('',*,*,#56334,.F.);
#80065=ORIENTED_EDGE('',*,*,#56796,.T.);
#80066=ORIENTED_EDGE('',*,*,#54919,.F.);
#80067=ORIENTED_EDGE('',*,*,#56798,.F.);
#80068=ORIENTED_EDGE('',*,*,#52540,.F.);
#80069=ORIENTED_EDGE('',*,*,#56797,.T.);
#80070=ORIENTED_EDGE('',*,*,#52122,.F.);
#80071=ORIENTED_EDGE('',*,*,#56799,.F.);
#80072=ORIENTED_EDGE('',*,*,#54907,.F.);
#80073=ORIENTED_EDGE('',*,*,#56798,.T.);
#80074=ORIENTED_EDGE('',*,*,#56333,.F.);
#80075=ORIENTED_EDGE('',*,*,#56800,.F.);
#80076=ORIENTED_EDGE('',*,*,#52541,.F.);
#80077=ORIENTED_EDGE('',*,*,#56799,.T.);
#80078=ORIENTED_EDGE('',*,*,#54312,.F.);
#80079=ORIENTED_EDGE('',*,*,#56801,.F.);
#80080=ORIENTED_EDGE('',*,*,#54908,.F.);
#80081=ORIENTED_EDGE('',*,*,#56800,.T.);
#80082=ORIENTED_EDGE('',*,*,#54903,.F.);
#80083=ORIENTED_EDGE('',*,*,#56802,.F.);
#80084=ORIENTED_EDGE('',*,*,#52542,.F.);
#80085=ORIENTED_EDGE('',*,*,#54307,.F.);
#80086=ORIENTED_EDGE('',*,*,#54303,.T.);
#80087=ORIENTED_EDGE('',*,*,#56803,.F.);
#80088=ORIENTED_EDGE('',*,*,#54909,.F.);
#80089=ORIENTED_EDGE('',*,*,#56801,.T.);
#80090=ORIENTED_EDGE('',*,*,#56802,.T.);
#80091=ORIENTED_EDGE('',*,*,#56335,.F.);
#80092=ORIENTED_EDGE('',*,*,#56804,.F.);
#80093=ORIENTED_EDGE('',*,*,#52543,.F.);
#80094=ORIENTED_EDGE('',*,*,#56803,.T.);
#80095=ORIENTED_EDGE('',*,*,#54302,.F.);
#80096=ORIENTED_EDGE('',*,*,#56805,.F.);
#80097=ORIENTED_EDGE('',*,*,#54910,.F.);
#80098=ORIENTED_EDGE('',*,*,#56804,.T.);
#80099=ORIENTED_EDGE('',*,*,#54905,.F.);
#80100=ORIENTED_EDGE('',*,*,#56806,.F.);
#80101=ORIENTED_EDGE('',*,*,#52544,.F.);
#80102=ORIENTED_EDGE('',*,*,#56805,.T.);
#80103=ORIENTED_EDGE('',*,*,#54314,.F.);
#80104=ORIENTED_EDGE('',*,*,#56807,.F.);
#80105=ORIENTED_EDGE('',*,*,#54911,.F.);
#80106=ORIENTED_EDGE('',*,*,#56806,.T.);
#80107=ORIENTED_EDGE('',*,*,#54904,.F.);
#80108=ORIENTED_EDGE('',*,*,#56808,.F.);
#80109=ORIENTED_EDGE('',*,*,#54310,.F.);
#80110=ORIENTED_EDGE('',*,*,#56807,.T.);
#80111=ORIENTED_EDGE('',*,*,#54298,.F.);
#80112=ORIENTED_EDGE('',*,*,#56809,.F.);
#80113=ORIENTED_EDGE('',*,*,#54912,.F.);
#80114=ORIENTED_EDGE('',*,*,#56808,.T.);
#80115=ORIENTED_EDGE('',*,*,#54915,.F.);
#80116=ORIENTED_EDGE('',*,*,#56810,.F.);
#80117=ORIENTED_EDGE('',*,*,#54289,.F.);
#80118=ORIENTED_EDGE('',*,*,#56809,.T.);
#80119=ORIENTED_EDGE('',*,*,#54316,.F.);
#80120=ORIENTED_EDGE('',*,*,#56811,.F.);
#80121=ORIENTED_EDGE('',*,*,#54913,.F.);
#80122=ORIENTED_EDGE('',*,*,#56810,.T.);
#80123=ORIENTED_EDGE('',*,*,#54914,.F.);
#80124=ORIENTED_EDGE('',*,*,#56811,.T.);
#80125=ORIENTED_EDGE('',*,*,#54294,.F.);
#80126=ORIENTED_EDGE('',*,*,#54290,.T.);
#80127=ORIENTED_EDGE('',*,*,#56812,.F.);
#80128=ORIENTED_EDGE('',*,*,#54954,.F.);
#80129=ORIENTED_EDGE('',*,*,#56813,.F.);
#80130=ORIENTED_EDGE('',*,*,#54246,.F.);
#80131=ORIENTED_EDGE('',*,*,#56813,.T.);
#80132=ORIENTED_EDGE('',*,*,#54953,.F.);
#80133=ORIENTED_EDGE('',*,*,#56814,.F.);
#80134=ORIENTED_EDGE('',*,*,#54255,.F.);
#80135=ORIENTED_EDGE('',*,*,#54245,.T.);
#80136=ORIENTED_EDGE('',*,*,#54249,.F.);
#80137=ORIENTED_EDGE('',*,*,#56815,.F.);
#80138=ORIENTED_EDGE('',*,*,#54955,.F.);
#80139=ORIENTED_EDGE('',*,*,#56812,.T.);
#80140=ORIENTED_EDGE('',*,*,#56814,.T.);
#80141=ORIENTED_EDGE('',*,*,#54952,.F.);
#80142=ORIENTED_EDGE('',*,*,#56816,.F.);
#80143=ORIENTED_EDGE('',*,*,#54240,.F.);
#80144=ORIENTED_EDGE('',*,*,#56815,.T.);
#80145=ORIENTED_EDGE('',*,*,#54253,.F.);
#80146=ORIENTED_EDGE('',*,*,#56817,.F.);
#80147=ORIENTED_EDGE('',*,*,#54944,.F.);
#80148=ORIENTED_EDGE('',*,*,#56816,.T.);
#80149=ORIENTED_EDGE('',*,*,#54951,.F.);
#80150=ORIENTED_EDGE('',*,*,#56818,.F.);
#80151=ORIENTED_EDGE('',*,*,#54257,.F.);
#80152=ORIENTED_EDGE('',*,*,#56817,.T.);
#80153=ORIENTED_EDGE('',*,*,#52132,.F.);
#80154=ORIENTED_EDGE('',*,*,#56819,.F.);
#80155=ORIENTED_EDGE('',*,*,#54945,.F.);
#80156=ORIENTED_EDGE('',*,*,#56818,.T.);
#80157=ORIENTED_EDGE('',*,*,#54950,.F.);
#80158=ORIENTED_EDGE('',*,*,#56820,.F.);
#80159=ORIENTED_EDGE('',*,*,#54232,.T.);
#80160=ORIENTED_EDGE('',*,*,#54236,.F.);
#80161=ORIENTED_EDGE('',*,*,#56819,.T.);
#80162=ORIENTED_EDGE('',*,*,#52131,.F.);
#80163=ORIENTED_EDGE('',*,*,#56821,.F.);
#80164=ORIENTED_EDGE('',*,*,#56336,.F.);
#80165=ORIENTED_EDGE('',*,*,#56820,.T.);
#80166=ORIENTED_EDGE('',*,*,#54949,.F.);
#80167=ORIENTED_EDGE('',*,*,#56822,.F.);
#80168=ORIENTED_EDGE('',*,*,#54233,.F.);
#80169=ORIENTED_EDGE('',*,*,#56821,.T.);
#80170=ORIENTED_EDGE('',*,*,#52130,.F.);
#80171=ORIENTED_EDGE('',*,*,#56823,.F.);
#80172=ORIENTED_EDGE('',*,*,#54929,.F.);
#80173=ORIENTED_EDGE('',*,*,#56822,.T.);
#80174=ORIENTED_EDGE('',*,*,#54948,.F.);
#80175=ORIENTED_EDGE('',*,*,#56824,.F.);
#80176=ORIENTED_EDGE('',*,*,#54251,.F.);
#80177=ORIENTED_EDGE('',*,*,#56823,.T.);
#80178=ORIENTED_EDGE('',*,*,#52129,.F.);
#80179=ORIENTED_EDGE('',*,*,#56825,.F.);
#80180=ORIENTED_EDGE('',*,*,#56338,.F.);
#80181=ORIENTED_EDGE('',*,*,#56824,.T.);
#80182=ORIENTED_EDGE('',*,*,#54947,.F.);
#80183=ORIENTED_EDGE('',*,*,#56826,.F.);
#80184=ORIENTED_EDGE('',*,*,#52534,.F.);
#80185=ORIENTED_EDGE('',*,*,#56825,.T.);
#80186=ORIENTED_EDGE('',*,*,#52128,.F.);
#80187=ORIENTED_EDGE('',*,*,#56827,.F.);
#80188=ORIENTED_EDGE('',*,*,#54935,.F.);
#80189=ORIENTED_EDGE('',*,*,#56826,.T.);
#80190=ORIENTED_EDGE('',*,*,#56337,.F.);
#80191=ORIENTED_EDGE('',*,*,#56828,.F.);
#80192=ORIENTED_EDGE('',*,*,#52535,.F.);
#80193=ORIENTED_EDGE('',*,*,#56827,.T.);
#80194=ORIENTED_EDGE('',*,*,#54282,.F.);
#80195=ORIENTED_EDGE('',*,*,#56829,.F.);
#80196=ORIENTED_EDGE('',*,*,#54936,.F.);
#80197=ORIENTED_EDGE('',*,*,#56828,.T.);
#80198=ORIENTED_EDGE('',*,*,#54931,.F.);
#80199=ORIENTED_EDGE('',*,*,#56830,.F.);
#80200=ORIENTED_EDGE('',*,*,#52536,.F.);
#80201=ORIENTED_EDGE('',*,*,#54277,.F.);
#80202=ORIENTED_EDGE('',*,*,#54273,.T.);
#80203=ORIENTED_EDGE('',*,*,#56831,.F.);
#80204=ORIENTED_EDGE('',*,*,#54937,.F.);
#80205=ORIENTED_EDGE('',*,*,#56829,.T.);
#80206=ORIENTED_EDGE('',*,*,#56830,.T.);
#80207=ORIENTED_EDGE('',*,*,#56339,.F.);
#80208=ORIENTED_EDGE('',*,*,#56832,.F.);
#80209=ORIENTED_EDGE('',*,*,#52537,.F.);
#80210=ORIENTED_EDGE('',*,*,#56831,.T.);
#80211=ORIENTED_EDGE('',*,*,#54272,.F.);
#80212=ORIENTED_EDGE('',*,*,#56833,.F.);
#80213=ORIENTED_EDGE('',*,*,#54938,.F.);
#80214=ORIENTED_EDGE('',*,*,#56832,.T.);
#80215=ORIENTED_EDGE('',*,*,#54933,.F.);
#80216=ORIENTED_EDGE('',*,*,#56834,.F.);
#80217=ORIENTED_EDGE('',*,*,#52538,.F.);
#80218=ORIENTED_EDGE('',*,*,#56833,.T.);
#80219=ORIENTED_EDGE('',*,*,#54284,.F.);
#80220=ORIENTED_EDGE('',*,*,#56835,.F.);
#80221=ORIENTED_EDGE('',*,*,#54939,.F.);
#80222=ORIENTED_EDGE('',*,*,#56834,.T.);
#80223=ORIENTED_EDGE('',*,*,#54932,.F.);
#80224=ORIENTED_EDGE('',*,*,#56836,.F.);
#80225=ORIENTED_EDGE('',*,*,#54280,.F.);
#80226=ORIENTED_EDGE('',*,*,#56835,.T.);
#80227=ORIENTED_EDGE('',*,*,#54268,.F.);
#80228=ORIENTED_EDGE('',*,*,#56837,.F.);
#80229=ORIENTED_EDGE('',*,*,#54940,.F.);
#80230=ORIENTED_EDGE('',*,*,#56836,.T.);
#80231=ORIENTED_EDGE('',*,*,#54943,.F.);
#80232=ORIENTED_EDGE('',*,*,#56838,.F.);
#80233=ORIENTED_EDGE('',*,*,#54259,.F.);
#80234=ORIENTED_EDGE('',*,*,#56837,.T.);
#80235=ORIENTED_EDGE('',*,*,#54286,.F.);
#80236=ORIENTED_EDGE('',*,*,#56839,.F.);
#80237=ORIENTED_EDGE('',*,*,#54941,.F.);
#80238=ORIENTED_EDGE('',*,*,#56838,.T.);
#80239=ORIENTED_EDGE('',*,*,#54942,.F.);
#80240=ORIENTED_EDGE('',*,*,#56839,.T.);
#80241=ORIENTED_EDGE('',*,*,#54264,.F.);
#80242=ORIENTED_EDGE('',*,*,#54260,.T.);
#80243=ORIENTED_EDGE('',*,*,#56840,.F.);
#80244=ORIENTED_EDGE('',*,*,#54982,.F.);
#80245=ORIENTED_EDGE('',*,*,#56841,.F.);
#80246=ORIENTED_EDGE('',*,*,#54216,.F.);
#80247=ORIENTED_EDGE('',*,*,#56841,.T.);
#80248=ORIENTED_EDGE('',*,*,#54981,.F.);
#80249=ORIENTED_EDGE('',*,*,#56842,.F.);
#80250=ORIENTED_EDGE('',*,*,#54225,.F.);
#80251=ORIENTED_EDGE('',*,*,#54215,.T.);
#80252=ORIENTED_EDGE('',*,*,#54219,.F.);
#80253=ORIENTED_EDGE('',*,*,#56843,.F.);
#80254=ORIENTED_EDGE('',*,*,#54983,.F.);
#80255=ORIENTED_EDGE('',*,*,#56840,.T.);
#80256=ORIENTED_EDGE('',*,*,#56842,.T.);
#80257=ORIENTED_EDGE('',*,*,#54980,.F.);
#80258=ORIENTED_EDGE('',*,*,#56844,.F.);
#80259=ORIENTED_EDGE('',*,*,#54210,.F.);
#80260=ORIENTED_EDGE('',*,*,#56843,.T.);
#80261=ORIENTED_EDGE('',*,*,#54223,.F.);
#80262=ORIENTED_EDGE('',*,*,#56845,.F.);
#80263=ORIENTED_EDGE('',*,*,#54972,.F.);
#80264=ORIENTED_EDGE('',*,*,#56844,.T.);
#80265=ORIENTED_EDGE('',*,*,#54979,.F.);
#80266=ORIENTED_EDGE('',*,*,#56846,.F.);
#80267=ORIENTED_EDGE('',*,*,#54227,.F.);
#80268=ORIENTED_EDGE('',*,*,#56845,.T.);
#80269=ORIENTED_EDGE('',*,*,#52138,.F.);
#80270=ORIENTED_EDGE('',*,*,#56847,.F.);
#80271=ORIENTED_EDGE('',*,*,#54973,.F.);
#80272=ORIENTED_EDGE('',*,*,#56846,.T.);
#80273=ORIENTED_EDGE('',*,*,#54978,.F.);
#80274=ORIENTED_EDGE('',*,*,#56848,.F.);
#80275=ORIENTED_EDGE('',*,*,#54202,.T.);
#80276=ORIENTED_EDGE('',*,*,#54206,.F.);
#80277=ORIENTED_EDGE('',*,*,#56847,.T.);
#80278=ORIENTED_EDGE('',*,*,#52137,.F.);
#80279=ORIENTED_EDGE('',*,*,#56849,.F.);
#80280=ORIENTED_EDGE('',*,*,#56340,.F.);
#80281=ORIENTED_EDGE('',*,*,#56848,.T.);
#80282=ORIENTED_EDGE('',*,*,#54977,.F.);
#80283=ORIENTED_EDGE('',*,*,#56850,.F.);
#80284=ORIENTED_EDGE('',*,*,#54203,.F.);
#80285=ORIENTED_EDGE('',*,*,#56849,.T.);
#80286=ORIENTED_EDGE('',*,*,#52136,.F.);
#80287=ORIENTED_EDGE('',*,*,#56851,.F.);
#80288=ORIENTED_EDGE('',*,*,#54957,.F.);
#80289=ORIENTED_EDGE('',*,*,#56850,.T.);
#80290=ORIENTED_EDGE('',*,*,#54976,.F.);
#80291=ORIENTED_EDGE('',*,*,#56852,.F.);
#80292=ORIENTED_EDGE('',*,*,#54221,.F.);
#80293=ORIENTED_EDGE('',*,*,#56851,.T.);
#80294=ORIENTED_EDGE('',*,*,#52135,.F.);
#80295=ORIENTED_EDGE('',*,*,#56853,.F.);
#80296=ORIENTED_EDGE('',*,*,#56342,.F.);
#80297=ORIENTED_EDGE('',*,*,#56852,.T.);
#80298=ORIENTED_EDGE('',*,*,#54975,.F.);
#80299=ORIENTED_EDGE('',*,*,#56854,.F.);
#80300=ORIENTED_EDGE('',*,*,#52528,.F.);
#80301=ORIENTED_EDGE('',*,*,#56853,.T.);
#80302=ORIENTED_EDGE('',*,*,#52134,.F.);
#80303=ORIENTED_EDGE('',*,*,#56855,.F.);
#80304=ORIENTED_EDGE('',*,*,#54963,.F.);
#80305=ORIENTED_EDGE('',*,*,#56854,.T.);
#80306=ORIENTED_EDGE('',*,*,#56341,.F.);
#80307=ORIENTED_EDGE('',*,*,#56856,.F.);
#80308=ORIENTED_EDGE('',*,*,#52529,.F.);
#80309=ORIENTED_EDGE('',*,*,#56855,.T.);
#80310=ORIENTED_EDGE('',*,*,#54252,.F.);
#80311=ORIENTED_EDGE('',*,*,#56857,.F.);
#80312=ORIENTED_EDGE('',*,*,#54964,.F.);
#80313=ORIENTED_EDGE('',*,*,#56856,.T.);
#80314=ORIENTED_EDGE('',*,*,#54959,.F.);
#80315=ORIENTED_EDGE('',*,*,#56858,.F.);
#80316=ORIENTED_EDGE('',*,*,#52530,.F.);
#80317=ORIENTED_EDGE('',*,*,#54247,.F.);
#80318=ORIENTED_EDGE('',*,*,#54243,.T.);
#80319=ORIENTED_EDGE('',*,*,#56859,.F.);
#80320=ORIENTED_EDGE('',*,*,#54965,.F.);
#80321=ORIENTED_EDGE('',*,*,#56857,.T.);
#80322=ORIENTED_EDGE('',*,*,#56858,.T.);
#80323=ORIENTED_EDGE('',*,*,#56343,.F.);
#80324=ORIENTED_EDGE('',*,*,#56860,.F.);
#80325=ORIENTED_EDGE('',*,*,#52531,.F.);
#80326=ORIENTED_EDGE('',*,*,#56859,.T.);
#80327=ORIENTED_EDGE('',*,*,#54242,.F.);
#80328=ORIENTED_EDGE('',*,*,#56861,.F.);
#80329=ORIENTED_EDGE('',*,*,#54966,.F.);
#80330=ORIENTED_EDGE('',*,*,#56860,.T.);
#80331=ORIENTED_EDGE('',*,*,#54961,.F.);
#80332=ORIENTED_EDGE('',*,*,#56862,.F.);
#80333=ORIENTED_EDGE('',*,*,#52532,.F.);
#80334=ORIENTED_EDGE('',*,*,#56861,.T.);
#80335=ORIENTED_EDGE('',*,*,#54254,.F.);
#80336=ORIENTED_EDGE('',*,*,#56863,.F.);
#80337=ORIENTED_EDGE('',*,*,#54967,.F.);
#80338=ORIENTED_EDGE('',*,*,#56862,.T.);
#80339=ORIENTED_EDGE('',*,*,#54960,.F.);
#80340=ORIENTED_EDGE('',*,*,#56864,.F.);
#80341=ORIENTED_EDGE('',*,*,#54250,.F.);
#80342=ORIENTED_EDGE('',*,*,#56863,.T.);
#80343=ORIENTED_EDGE('',*,*,#54238,.F.);
#80344=ORIENTED_EDGE('',*,*,#56865,.F.);
#80345=ORIENTED_EDGE('',*,*,#54968,.F.);
#80346=ORIENTED_EDGE('',*,*,#56864,.T.);
#80347=ORIENTED_EDGE('',*,*,#54971,.F.);
#80348=ORIENTED_EDGE('',*,*,#56866,.F.);
#80349=ORIENTED_EDGE('',*,*,#54229,.F.);
#80350=ORIENTED_EDGE('',*,*,#56865,.T.);
#80351=ORIENTED_EDGE('',*,*,#54256,.F.);
#80352=ORIENTED_EDGE('',*,*,#56867,.F.);
#80353=ORIENTED_EDGE('',*,*,#54969,.F.);
#80354=ORIENTED_EDGE('',*,*,#56866,.T.);
#80355=ORIENTED_EDGE('',*,*,#54970,.F.);
#80356=ORIENTED_EDGE('',*,*,#56867,.T.);
#80357=ORIENTED_EDGE('',*,*,#54234,.F.);
#80358=ORIENTED_EDGE('',*,*,#54230,.T.);
#80359=ORIENTED_EDGE('',*,*,#56868,.F.);
#80360=ORIENTED_EDGE('',*,*,#55010,.F.);
#80361=ORIENTED_EDGE('',*,*,#56869,.F.);
#80362=ORIENTED_EDGE('',*,*,#54186,.F.);
#80363=ORIENTED_EDGE('',*,*,#56869,.T.);
#80364=ORIENTED_EDGE('',*,*,#55009,.F.);
#80365=ORIENTED_EDGE('',*,*,#56870,.F.);
#80366=ORIENTED_EDGE('',*,*,#54195,.F.);
#80367=ORIENTED_EDGE('',*,*,#54185,.T.);
#80368=ORIENTED_EDGE('',*,*,#54189,.F.);
#80369=ORIENTED_EDGE('',*,*,#56871,.F.);
#80370=ORIENTED_EDGE('',*,*,#55011,.F.);
#80371=ORIENTED_EDGE('',*,*,#56868,.T.);
#80372=ORIENTED_EDGE('',*,*,#56870,.T.);
#80373=ORIENTED_EDGE('',*,*,#55008,.F.);
#80374=ORIENTED_EDGE('',*,*,#56872,.F.);
#80375=ORIENTED_EDGE('',*,*,#54180,.F.);
#80376=ORIENTED_EDGE('',*,*,#56871,.T.);
#80377=ORIENTED_EDGE('',*,*,#54193,.F.);
#80378=ORIENTED_EDGE('',*,*,#56873,.F.);
#80379=ORIENTED_EDGE('',*,*,#55000,.F.);
#80380=ORIENTED_EDGE('',*,*,#56872,.T.);
#80381=ORIENTED_EDGE('',*,*,#55007,.F.);
#80382=ORIENTED_EDGE('',*,*,#56874,.F.);
#80383=ORIENTED_EDGE('',*,*,#54197,.F.);
#80384=ORIENTED_EDGE('',*,*,#56873,.T.);
#80385=ORIENTED_EDGE('',*,*,#52144,.F.);
#80386=ORIENTED_EDGE('',*,*,#56875,.F.);
#80387=ORIENTED_EDGE('',*,*,#55001,.F.);
#80388=ORIENTED_EDGE('',*,*,#56874,.T.);
#80389=ORIENTED_EDGE('',*,*,#55006,.F.);
#80390=ORIENTED_EDGE('',*,*,#56876,.F.);
#80391=ORIENTED_EDGE('',*,*,#54172,.T.);
#80392=ORIENTED_EDGE('',*,*,#54176,.F.);
#80393=ORIENTED_EDGE('',*,*,#56875,.T.);
#80394=ORIENTED_EDGE('',*,*,#52143,.F.);
#80395=ORIENTED_EDGE('',*,*,#56877,.F.);
#80396=ORIENTED_EDGE('',*,*,#56344,.F.);
#80397=ORIENTED_EDGE('',*,*,#56876,.T.);
#80398=ORIENTED_EDGE('',*,*,#55005,.F.);
#80399=ORIENTED_EDGE('',*,*,#56878,.F.);
#80400=ORIENTED_EDGE('',*,*,#54173,.F.);
#80401=ORIENTED_EDGE('',*,*,#56877,.T.);
#80402=ORIENTED_EDGE('',*,*,#52142,.F.);
#80403=ORIENTED_EDGE('',*,*,#56879,.F.);
#80404=ORIENTED_EDGE('',*,*,#54985,.F.);
#80405=ORIENTED_EDGE('',*,*,#56878,.T.);
#80406=ORIENTED_EDGE('',*,*,#55004,.F.);
#80407=ORIENTED_EDGE('',*,*,#56880,.F.);
#80408=ORIENTED_EDGE('',*,*,#54191,.F.);
#80409=ORIENTED_EDGE('',*,*,#56879,.T.);
#80410=ORIENTED_EDGE('',*,*,#52141,.F.);
#80411=ORIENTED_EDGE('',*,*,#56881,.F.);
#80412=ORIENTED_EDGE('',*,*,#56346,.F.);
#80413=ORIENTED_EDGE('',*,*,#56880,.T.);
#80414=ORIENTED_EDGE('',*,*,#55003,.F.);
#80415=ORIENTED_EDGE('',*,*,#56882,.F.);
#80416=ORIENTED_EDGE('',*,*,#52522,.F.);
#80417=ORIENTED_EDGE('',*,*,#56881,.T.);
#80418=ORIENTED_EDGE('',*,*,#52140,.F.);
#80419=ORIENTED_EDGE('',*,*,#56883,.F.);
#80420=ORIENTED_EDGE('',*,*,#54991,.F.);
#80421=ORIENTED_EDGE('',*,*,#56882,.T.);
#80422=ORIENTED_EDGE('',*,*,#56345,.F.);
#80423=ORIENTED_EDGE('',*,*,#56884,.F.);
#80424=ORIENTED_EDGE('',*,*,#52523,.F.);
#80425=ORIENTED_EDGE('',*,*,#56883,.T.);
#80426=ORIENTED_EDGE('',*,*,#54222,.F.);
#80427=ORIENTED_EDGE('',*,*,#56885,.F.);
#80428=ORIENTED_EDGE('',*,*,#54992,.F.);
#80429=ORIENTED_EDGE('',*,*,#56884,.T.);
#80430=ORIENTED_EDGE('',*,*,#54987,.F.);
#80431=ORIENTED_EDGE('',*,*,#56886,.F.);
#80432=ORIENTED_EDGE('',*,*,#52524,.F.);
#80433=ORIENTED_EDGE('',*,*,#54217,.F.);
#80434=ORIENTED_EDGE('',*,*,#54213,.T.);
#80435=ORIENTED_EDGE('',*,*,#56887,.F.);
#80436=ORIENTED_EDGE('',*,*,#54993,.F.);
#80437=ORIENTED_EDGE('',*,*,#56885,.T.);
#80438=ORIENTED_EDGE('',*,*,#56886,.T.);
#80439=ORIENTED_EDGE('',*,*,#56347,.F.);
#80440=ORIENTED_EDGE('',*,*,#56888,.F.);
#80441=ORIENTED_EDGE('',*,*,#52525,.F.);
#80442=ORIENTED_EDGE('',*,*,#56887,.T.);
#80443=ORIENTED_EDGE('',*,*,#54212,.F.);
#80444=ORIENTED_EDGE('',*,*,#56889,.F.);
#80445=ORIENTED_EDGE('',*,*,#54994,.F.);
#80446=ORIENTED_EDGE('',*,*,#56888,.T.);
#80447=ORIENTED_EDGE('',*,*,#54989,.F.);
#80448=ORIENTED_EDGE('',*,*,#56890,.F.);
#80449=ORIENTED_EDGE('',*,*,#52526,.F.);
#80450=ORIENTED_EDGE('',*,*,#56889,.T.);
#80451=ORIENTED_EDGE('',*,*,#54224,.F.);
#80452=ORIENTED_EDGE('',*,*,#56891,.F.);
#80453=ORIENTED_EDGE('',*,*,#54995,.F.);
#80454=ORIENTED_EDGE('',*,*,#56890,.T.);
#80455=ORIENTED_EDGE('',*,*,#54988,.F.);
#80456=ORIENTED_EDGE('',*,*,#56892,.F.);
#80457=ORIENTED_EDGE('',*,*,#54220,.F.);
#80458=ORIENTED_EDGE('',*,*,#56891,.T.);
#80459=ORIENTED_EDGE('',*,*,#54208,.F.);
#80460=ORIENTED_EDGE('',*,*,#56893,.F.);
#80461=ORIENTED_EDGE('',*,*,#54996,.F.);
#80462=ORIENTED_EDGE('',*,*,#56892,.T.);
#80463=ORIENTED_EDGE('',*,*,#54999,.F.);
#80464=ORIENTED_EDGE('',*,*,#56894,.F.);
#80465=ORIENTED_EDGE('',*,*,#54199,.F.);
#80466=ORIENTED_EDGE('',*,*,#56893,.T.);
#80467=ORIENTED_EDGE('',*,*,#54226,.F.);
#80468=ORIENTED_EDGE('',*,*,#56895,.F.);
#80469=ORIENTED_EDGE('',*,*,#54997,.F.);
#80470=ORIENTED_EDGE('',*,*,#56894,.T.);
#80471=ORIENTED_EDGE('',*,*,#54998,.F.);
#80472=ORIENTED_EDGE('',*,*,#56895,.T.);
#80473=ORIENTED_EDGE('',*,*,#54204,.F.);
#80474=ORIENTED_EDGE('',*,*,#54200,.T.);
#80475=ORIENTED_EDGE('',*,*,#56896,.F.);
#80476=ORIENTED_EDGE('',*,*,#55038,.F.);
#80477=ORIENTED_EDGE('',*,*,#56897,.F.);
#80478=ORIENTED_EDGE('',*,*,#54156,.F.);
#80479=ORIENTED_EDGE('',*,*,#56897,.T.);
#80480=ORIENTED_EDGE('',*,*,#55037,.F.);
#80481=ORIENTED_EDGE('',*,*,#56898,.F.);
#80482=ORIENTED_EDGE('',*,*,#54165,.F.);
#80483=ORIENTED_EDGE('',*,*,#54155,.T.);
#80484=ORIENTED_EDGE('',*,*,#54159,.F.);
#80485=ORIENTED_EDGE('',*,*,#56899,.F.);
#80486=ORIENTED_EDGE('',*,*,#55039,.F.);
#80487=ORIENTED_EDGE('',*,*,#56896,.T.);
#80488=ORIENTED_EDGE('',*,*,#56898,.T.);
#80489=ORIENTED_EDGE('',*,*,#55036,.F.);
#80490=ORIENTED_EDGE('',*,*,#56900,.F.);
#80491=ORIENTED_EDGE('',*,*,#54150,.F.);
#80492=ORIENTED_EDGE('',*,*,#56899,.T.);
#80493=ORIENTED_EDGE('',*,*,#54163,.F.);
#80494=ORIENTED_EDGE('',*,*,#56901,.F.);
#80495=ORIENTED_EDGE('',*,*,#55028,.F.);
#80496=ORIENTED_EDGE('',*,*,#56900,.T.);
#80497=ORIENTED_EDGE('',*,*,#55035,.F.);
#80498=ORIENTED_EDGE('',*,*,#56902,.F.);
#80499=ORIENTED_EDGE('',*,*,#54167,.F.);
#80500=ORIENTED_EDGE('',*,*,#56901,.T.);
#80501=ORIENTED_EDGE('',*,*,#52150,.F.);
#80502=ORIENTED_EDGE('',*,*,#56903,.F.);
#80503=ORIENTED_EDGE('',*,*,#55029,.F.);
#80504=ORIENTED_EDGE('',*,*,#56902,.T.);
#80505=ORIENTED_EDGE('',*,*,#55034,.F.);
#80506=ORIENTED_EDGE('',*,*,#56904,.F.);
#80507=ORIENTED_EDGE('',*,*,#54142,.T.);
#80508=ORIENTED_EDGE('',*,*,#54146,.F.);
#80509=ORIENTED_EDGE('',*,*,#56903,.T.);
#80510=ORIENTED_EDGE('',*,*,#52149,.F.);
#80511=ORIENTED_EDGE('',*,*,#56905,.F.);
#80512=ORIENTED_EDGE('',*,*,#56348,.F.);
#80513=ORIENTED_EDGE('',*,*,#56904,.T.);
#80514=ORIENTED_EDGE('',*,*,#55033,.F.);
#80515=ORIENTED_EDGE('',*,*,#56906,.F.);
#80516=ORIENTED_EDGE('',*,*,#54143,.F.);
#80517=ORIENTED_EDGE('',*,*,#56905,.T.);
#80518=ORIENTED_EDGE('',*,*,#52148,.F.);
#80519=ORIENTED_EDGE('',*,*,#56907,.F.);
#80520=ORIENTED_EDGE('',*,*,#55013,.F.);
#80521=ORIENTED_EDGE('',*,*,#56906,.T.);
#80522=ORIENTED_EDGE('',*,*,#55032,.F.);
#80523=ORIENTED_EDGE('',*,*,#56908,.F.);
#80524=ORIENTED_EDGE('',*,*,#54161,.F.);
#80525=ORIENTED_EDGE('',*,*,#56907,.T.);
#80526=ORIENTED_EDGE('',*,*,#52147,.F.);
#80527=ORIENTED_EDGE('',*,*,#56909,.F.);
#80528=ORIENTED_EDGE('',*,*,#56350,.F.);
#80529=ORIENTED_EDGE('',*,*,#56908,.T.);
#80530=ORIENTED_EDGE('',*,*,#55031,.F.);
#80531=ORIENTED_EDGE('',*,*,#56910,.F.);
#80532=ORIENTED_EDGE('',*,*,#52516,.F.);
#80533=ORIENTED_EDGE('',*,*,#56909,.T.);
#80534=ORIENTED_EDGE('',*,*,#52146,.F.);
#80535=ORIENTED_EDGE('',*,*,#56911,.F.);
#80536=ORIENTED_EDGE('',*,*,#55019,.F.);
#80537=ORIENTED_EDGE('',*,*,#56910,.T.);
#80538=ORIENTED_EDGE('',*,*,#56349,.F.);
#80539=ORIENTED_EDGE('',*,*,#56912,.F.);
#80540=ORIENTED_EDGE('',*,*,#52517,.F.);
#80541=ORIENTED_EDGE('',*,*,#56911,.T.);
#80542=ORIENTED_EDGE('',*,*,#54192,.F.);
#80543=ORIENTED_EDGE('',*,*,#56913,.F.);
#80544=ORIENTED_EDGE('',*,*,#55020,.F.);
#80545=ORIENTED_EDGE('',*,*,#56912,.T.);
#80546=ORIENTED_EDGE('',*,*,#55015,.F.);
#80547=ORIENTED_EDGE('',*,*,#56914,.F.);
#80548=ORIENTED_EDGE('',*,*,#52518,.F.);
#80549=ORIENTED_EDGE('',*,*,#54187,.F.);
#80550=ORIENTED_EDGE('',*,*,#54183,.T.);
#80551=ORIENTED_EDGE('',*,*,#56915,.F.);
#80552=ORIENTED_EDGE('',*,*,#55021,.F.);
#80553=ORIENTED_EDGE('',*,*,#56913,.T.);
#80554=ORIENTED_EDGE('',*,*,#56914,.T.);
#80555=ORIENTED_EDGE('',*,*,#56351,.F.);
#80556=ORIENTED_EDGE('',*,*,#56916,.F.);
#80557=ORIENTED_EDGE('',*,*,#52519,.F.);
#80558=ORIENTED_EDGE('',*,*,#56915,.T.);
#80559=ORIENTED_EDGE('',*,*,#54182,.F.);
#80560=ORIENTED_EDGE('',*,*,#56917,.F.);
#80561=ORIENTED_EDGE('',*,*,#55022,.F.);
#80562=ORIENTED_EDGE('',*,*,#56916,.T.);
#80563=ORIENTED_EDGE('',*,*,#55017,.F.);
#80564=ORIENTED_EDGE('',*,*,#56918,.F.);
#80565=ORIENTED_EDGE('',*,*,#52520,.F.);
#80566=ORIENTED_EDGE('',*,*,#56917,.T.);
#80567=ORIENTED_EDGE('',*,*,#54194,.F.);
#80568=ORIENTED_EDGE('',*,*,#56919,.F.);
#80569=ORIENTED_EDGE('',*,*,#55023,.F.);
#80570=ORIENTED_EDGE('',*,*,#56918,.T.);
#80571=ORIENTED_EDGE('',*,*,#55016,.F.);
#80572=ORIENTED_EDGE('',*,*,#56920,.F.);
#80573=ORIENTED_EDGE('',*,*,#54190,.F.);
#80574=ORIENTED_EDGE('',*,*,#56919,.T.);
#80575=ORIENTED_EDGE('',*,*,#54178,.F.);
#80576=ORIENTED_EDGE('',*,*,#56921,.F.);
#80577=ORIENTED_EDGE('',*,*,#55024,.F.);
#80578=ORIENTED_EDGE('',*,*,#56920,.T.);
#80579=ORIENTED_EDGE('',*,*,#55027,.F.);
#80580=ORIENTED_EDGE('',*,*,#56922,.F.);
#80581=ORIENTED_EDGE('',*,*,#54169,.F.);
#80582=ORIENTED_EDGE('',*,*,#56921,.T.);
#80583=ORIENTED_EDGE('',*,*,#54196,.F.);
#80584=ORIENTED_EDGE('',*,*,#56923,.F.);
#80585=ORIENTED_EDGE('',*,*,#55025,.F.);
#80586=ORIENTED_EDGE('',*,*,#56922,.T.);
#80587=ORIENTED_EDGE('',*,*,#55026,.F.);
#80588=ORIENTED_EDGE('',*,*,#56923,.T.);
#80589=ORIENTED_EDGE('',*,*,#54174,.F.);
#80590=ORIENTED_EDGE('',*,*,#54170,.T.);
#80591=ORIENTED_EDGE('',*,*,#56924,.F.);
#80592=ORIENTED_EDGE('',*,*,#55066,.F.);
#80593=ORIENTED_EDGE('',*,*,#56925,.F.);
#80594=ORIENTED_EDGE('',*,*,#54126,.F.);
#80595=ORIENTED_EDGE('',*,*,#56925,.T.);
#80596=ORIENTED_EDGE('',*,*,#55065,.F.);
#80597=ORIENTED_EDGE('',*,*,#56926,.F.);
#80598=ORIENTED_EDGE('',*,*,#54135,.F.);
#80599=ORIENTED_EDGE('',*,*,#54125,.T.);
#80600=ORIENTED_EDGE('',*,*,#54129,.F.);
#80601=ORIENTED_EDGE('',*,*,#56927,.F.);
#80602=ORIENTED_EDGE('',*,*,#55067,.F.);
#80603=ORIENTED_EDGE('',*,*,#56924,.T.);
#80604=ORIENTED_EDGE('',*,*,#56926,.T.);
#80605=ORIENTED_EDGE('',*,*,#55064,.F.);
#80606=ORIENTED_EDGE('',*,*,#56928,.F.);
#80607=ORIENTED_EDGE('',*,*,#54120,.F.);
#80608=ORIENTED_EDGE('',*,*,#56927,.T.);
#80609=ORIENTED_EDGE('',*,*,#54133,.F.);
#80610=ORIENTED_EDGE('',*,*,#56929,.F.);
#80611=ORIENTED_EDGE('',*,*,#55056,.F.);
#80612=ORIENTED_EDGE('',*,*,#56928,.T.);
#80613=ORIENTED_EDGE('',*,*,#55063,.F.);
#80614=ORIENTED_EDGE('',*,*,#56930,.F.);
#80615=ORIENTED_EDGE('',*,*,#54137,.F.);
#80616=ORIENTED_EDGE('',*,*,#56929,.T.);
#80617=ORIENTED_EDGE('',*,*,#52156,.F.);
#80618=ORIENTED_EDGE('',*,*,#56931,.F.);
#80619=ORIENTED_EDGE('',*,*,#55057,.F.);
#80620=ORIENTED_EDGE('',*,*,#56930,.T.);
#80621=ORIENTED_EDGE('',*,*,#55062,.F.);
#80622=ORIENTED_EDGE('',*,*,#56932,.F.);
#80623=ORIENTED_EDGE('',*,*,#54112,.T.);
#80624=ORIENTED_EDGE('',*,*,#54116,.F.);
#80625=ORIENTED_EDGE('',*,*,#56931,.T.);
#80626=ORIENTED_EDGE('',*,*,#52155,.F.);
#80627=ORIENTED_EDGE('',*,*,#56933,.F.);
#80628=ORIENTED_EDGE('',*,*,#56352,.F.);
#80629=ORIENTED_EDGE('',*,*,#56932,.T.);
#80630=ORIENTED_EDGE('',*,*,#55061,.F.);
#80631=ORIENTED_EDGE('',*,*,#56934,.F.);
#80632=ORIENTED_EDGE('',*,*,#54113,.F.);
#80633=ORIENTED_EDGE('',*,*,#56933,.T.);
#80634=ORIENTED_EDGE('',*,*,#52154,.F.);
#80635=ORIENTED_EDGE('',*,*,#56935,.F.);
#80636=ORIENTED_EDGE('',*,*,#55041,.F.);
#80637=ORIENTED_EDGE('',*,*,#56934,.T.);
#80638=ORIENTED_EDGE('',*,*,#55060,.F.);
#80639=ORIENTED_EDGE('',*,*,#56936,.F.);
#80640=ORIENTED_EDGE('',*,*,#54131,.F.);
#80641=ORIENTED_EDGE('',*,*,#56935,.T.);
#80642=ORIENTED_EDGE('',*,*,#52153,.F.);
#80643=ORIENTED_EDGE('',*,*,#56937,.F.);
#80644=ORIENTED_EDGE('',*,*,#56354,.F.);
#80645=ORIENTED_EDGE('',*,*,#56936,.T.);
#80646=ORIENTED_EDGE('',*,*,#55059,.F.);
#80647=ORIENTED_EDGE('',*,*,#56938,.F.);
#80648=ORIENTED_EDGE('',*,*,#52510,.F.);
#80649=ORIENTED_EDGE('',*,*,#56937,.T.);
#80650=ORIENTED_EDGE('',*,*,#52152,.F.);
#80651=ORIENTED_EDGE('',*,*,#56939,.F.);
#80652=ORIENTED_EDGE('',*,*,#55047,.F.);
#80653=ORIENTED_EDGE('',*,*,#56938,.T.);
#80654=ORIENTED_EDGE('',*,*,#56353,.F.);
#80655=ORIENTED_EDGE('',*,*,#56940,.F.);
#80656=ORIENTED_EDGE('',*,*,#52511,.F.);
#80657=ORIENTED_EDGE('',*,*,#56939,.T.);
#80658=ORIENTED_EDGE('',*,*,#54162,.F.);
#80659=ORIENTED_EDGE('',*,*,#56941,.F.);
#80660=ORIENTED_EDGE('',*,*,#55048,.F.);
#80661=ORIENTED_EDGE('',*,*,#56940,.T.);
#80662=ORIENTED_EDGE('',*,*,#55043,.F.);
#80663=ORIENTED_EDGE('',*,*,#56942,.F.);
#80664=ORIENTED_EDGE('',*,*,#52512,.F.);
#80665=ORIENTED_EDGE('',*,*,#54157,.F.);
#80666=ORIENTED_EDGE('',*,*,#54153,.T.);
#80667=ORIENTED_EDGE('',*,*,#56943,.F.);
#80668=ORIENTED_EDGE('',*,*,#55049,.F.);
#80669=ORIENTED_EDGE('',*,*,#56941,.T.);
#80670=ORIENTED_EDGE('',*,*,#56942,.T.);
#80671=ORIENTED_EDGE('',*,*,#56355,.F.);
#80672=ORIENTED_EDGE('',*,*,#56944,.F.);
#80673=ORIENTED_EDGE('',*,*,#52513,.F.);
#80674=ORIENTED_EDGE('',*,*,#56943,.T.);
#80675=ORIENTED_EDGE('',*,*,#54152,.F.);
#80676=ORIENTED_EDGE('',*,*,#56945,.F.);
#80677=ORIENTED_EDGE('',*,*,#55050,.F.);
#80678=ORIENTED_EDGE('',*,*,#56944,.T.);
#80679=ORIENTED_EDGE('',*,*,#55045,.F.);
#80680=ORIENTED_EDGE('',*,*,#56946,.F.);
#80681=ORIENTED_EDGE('',*,*,#52514,.F.);
#80682=ORIENTED_EDGE('',*,*,#56945,.T.);
#80683=ORIENTED_EDGE('',*,*,#54164,.F.);
#80684=ORIENTED_EDGE('',*,*,#56947,.F.);
#80685=ORIENTED_EDGE('',*,*,#55051,.F.);
#80686=ORIENTED_EDGE('',*,*,#56946,.T.);
#80687=ORIENTED_EDGE('',*,*,#55044,.F.);
#80688=ORIENTED_EDGE('',*,*,#56948,.F.);
#80689=ORIENTED_EDGE('',*,*,#54160,.F.);
#80690=ORIENTED_EDGE('',*,*,#56947,.T.);
#80691=ORIENTED_EDGE('',*,*,#54148,.F.);
#80692=ORIENTED_EDGE('',*,*,#56949,.F.);
#80693=ORIENTED_EDGE('',*,*,#55052,.F.);
#80694=ORIENTED_EDGE('',*,*,#56948,.T.);
#80695=ORIENTED_EDGE('',*,*,#55055,.F.);
#80696=ORIENTED_EDGE('',*,*,#56950,.F.);
#80697=ORIENTED_EDGE('',*,*,#54139,.F.);
#80698=ORIENTED_EDGE('',*,*,#56949,.T.);
#80699=ORIENTED_EDGE('',*,*,#54166,.F.);
#80700=ORIENTED_EDGE('',*,*,#56951,.F.);
#80701=ORIENTED_EDGE('',*,*,#55053,.F.);
#80702=ORIENTED_EDGE('',*,*,#56950,.T.);
#80703=ORIENTED_EDGE('',*,*,#55054,.F.);
#80704=ORIENTED_EDGE('',*,*,#56951,.T.);
#80705=ORIENTED_EDGE('',*,*,#54144,.F.);
#80706=ORIENTED_EDGE('',*,*,#54140,.T.);
#80707=ORIENTED_EDGE('',*,*,#56952,.F.);
#80708=ORIENTED_EDGE('',*,*,#55094,.F.);
#80709=ORIENTED_EDGE('',*,*,#56953,.F.);
#80710=ORIENTED_EDGE('',*,*,#54096,.F.);
#80711=ORIENTED_EDGE('',*,*,#56953,.T.);
#80712=ORIENTED_EDGE('',*,*,#55093,.F.);
#80713=ORIENTED_EDGE('',*,*,#56954,.F.);
#80714=ORIENTED_EDGE('',*,*,#54105,.F.);
#80715=ORIENTED_EDGE('',*,*,#54095,.T.);
#80716=ORIENTED_EDGE('',*,*,#54099,.F.);
#80717=ORIENTED_EDGE('',*,*,#56955,.F.);
#80718=ORIENTED_EDGE('',*,*,#55095,.F.);
#80719=ORIENTED_EDGE('',*,*,#56952,.T.);
#80720=ORIENTED_EDGE('',*,*,#56954,.T.);
#80721=ORIENTED_EDGE('',*,*,#55092,.F.);
#80722=ORIENTED_EDGE('',*,*,#56956,.F.);
#80723=ORIENTED_EDGE('',*,*,#54090,.F.);
#80724=ORIENTED_EDGE('',*,*,#56955,.T.);
#80725=ORIENTED_EDGE('',*,*,#54103,.F.);
#80726=ORIENTED_EDGE('',*,*,#56957,.F.);
#80727=ORIENTED_EDGE('',*,*,#55084,.F.);
#80728=ORIENTED_EDGE('',*,*,#56956,.T.);
#80729=ORIENTED_EDGE('',*,*,#55091,.F.);
#80730=ORIENTED_EDGE('',*,*,#56958,.F.);
#80731=ORIENTED_EDGE('',*,*,#54107,.F.);
#80732=ORIENTED_EDGE('',*,*,#56957,.T.);
#80733=ORIENTED_EDGE('',*,*,#52162,.F.);
#80734=ORIENTED_EDGE('',*,*,#56959,.F.);
#80735=ORIENTED_EDGE('',*,*,#55085,.F.);
#80736=ORIENTED_EDGE('',*,*,#56958,.T.);
#80737=ORIENTED_EDGE('',*,*,#55090,.F.);
#80738=ORIENTED_EDGE('',*,*,#56960,.F.);
#80739=ORIENTED_EDGE('',*,*,#54082,.T.);
#80740=ORIENTED_EDGE('',*,*,#54086,.F.);
#80741=ORIENTED_EDGE('',*,*,#56959,.T.);
#80742=ORIENTED_EDGE('',*,*,#52161,.F.);
#80743=ORIENTED_EDGE('',*,*,#56961,.F.);
#80744=ORIENTED_EDGE('',*,*,#56356,.F.);
#80745=ORIENTED_EDGE('',*,*,#56960,.T.);
#80746=ORIENTED_EDGE('',*,*,#55089,.F.);
#80747=ORIENTED_EDGE('',*,*,#56962,.F.);
#80748=ORIENTED_EDGE('',*,*,#54083,.F.);
#80749=ORIENTED_EDGE('',*,*,#56961,.T.);
#80750=ORIENTED_EDGE('',*,*,#52160,.F.);
#80751=ORIENTED_EDGE('',*,*,#56963,.F.);
#80752=ORIENTED_EDGE('',*,*,#55069,.F.);
#80753=ORIENTED_EDGE('',*,*,#56962,.T.);
#80754=ORIENTED_EDGE('',*,*,#55088,.F.);
#80755=ORIENTED_EDGE('',*,*,#56964,.F.);
#80756=ORIENTED_EDGE('',*,*,#54101,.F.);
#80757=ORIENTED_EDGE('',*,*,#56963,.T.);
#80758=ORIENTED_EDGE('',*,*,#52159,.F.);
#80759=ORIENTED_EDGE('',*,*,#56965,.F.);
#80760=ORIENTED_EDGE('',*,*,#56358,.F.);
#80761=ORIENTED_EDGE('',*,*,#56964,.T.);
#80762=ORIENTED_EDGE('',*,*,#55087,.F.);
#80763=ORIENTED_EDGE('',*,*,#56966,.F.);
#80764=ORIENTED_EDGE('',*,*,#52504,.F.);
#80765=ORIENTED_EDGE('',*,*,#56965,.T.);
#80766=ORIENTED_EDGE('',*,*,#52158,.F.);
#80767=ORIENTED_EDGE('',*,*,#56967,.F.);
#80768=ORIENTED_EDGE('',*,*,#55075,.F.);
#80769=ORIENTED_EDGE('',*,*,#56966,.T.);
#80770=ORIENTED_EDGE('',*,*,#56357,.F.);
#80771=ORIENTED_EDGE('',*,*,#56968,.F.);
#80772=ORIENTED_EDGE('',*,*,#52505,.F.);
#80773=ORIENTED_EDGE('',*,*,#56967,.T.);
#80774=ORIENTED_EDGE('',*,*,#54132,.F.);
#80775=ORIENTED_EDGE('',*,*,#56969,.F.);
#80776=ORIENTED_EDGE('',*,*,#55076,.F.);
#80777=ORIENTED_EDGE('',*,*,#56968,.T.);
#80778=ORIENTED_EDGE('',*,*,#55071,.F.);
#80779=ORIENTED_EDGE('',*,*,#56970,.F.);
#80780=ORIENTED_EDGE('',*,*,#52506,.F.);
#80781=ORIENTED_EDGE('',*,*,#54127,.F.);
#80782=ORIENTED_EDGE('',*,*,#54123,.T.);
#80783=ORIENTED_EDGE('',*,*,#56971,.F.);
#80784=ORIENTED_EDGE('',*,*,#55077,.F.);
#80785=ORIENTED_EDGE('',*,*,#56969,.T.);
#80786=ORIENTED_EDGE('',*,*,#56970,.T.);
#80787=ORIENTED_EDGE('',*,*,#56359,.F.);
#80788=ORIENTED_EDGE('',*,*,#56972,.F.);
#80789=ORIENTED_EDGE('',*,*,#52507,.F.);
#80790=ORIENTED_EDGE('',*,*,#56971,.T.);
#80791=ORIENTED_EDGE('',*,*,#54122,.F.);
#80792=ORIENTED_EDGE('',*,*,#56973,.F.);
#80793=ORIENTED_EDGE('',*,*,#55078,.F.);
#80794=ORIENTED_EDGE('',*,*,#56972,.T.);
#80795=ORIENTED_EDGE('',*,*,#55073,.F.);
#80796=ORIENTED_EDGE('',*,*,#56974,.F.);
#80797=ORIENTED_EDGE('',*,*,#52508,.F.);
#80798=ORIENTED_EDGE('',*,*,#56973,.T.);
#80799=ORIENTED_EDGE('',*,*,#54134,.F.);
#80800=ORIENTED_EDGE('',*,*,#56975,.F.);
#80801=ORIENTED_EDGE('',*,*,#55079,.F.);
#80802=ORIENTED_EDGE('',*,*,#56974,.T.);
#80803=ORIENTED_EDGE('',*,*,#55072,.F.);
#80804=ORIENTED_EDGE('',*,*,#56976,.F.);
#80805=ORIENTED_EDGE('',*,*,#54130,.F.);
#80806=ORIENTED_EDGE('',*,*,#56975,.T.);
#80807=ORIENTED_EDGE('',*,*,#54118,.F.);
#80808=ORIENTED_EDGE('',*,*,#56977,.F.);
#80809=ORIENTED_EDGE('',*,*,#55080,.F.);
#80810=ORIENTED_EDGE('',*,*,#56976,.T.);
#80811=ORIENTED_EDGE('',*,*,#55083,.F.);
#80812=ORIENTED_EDGE('',*,*,#56978,.F.);
#80813=ORIENTED_EDGE('',*,*,#54109,.F.);
#80814=ORIENTED_EDGE('',*,*,#56977,.T.);
#80815=ORIENTED_EDGE('',*,*,#54136,.F.);
#80816=ORIENTED_EDGE('',*,*,#56979,.F.);
#80817=ORIENTED_EDGE('',*,*,#55081,.F.);
#80818=ORIENTED_EDGE('',*,*,#56978,.T.);
#80819=ORIENTED_EDGE('',*,*,#55082,.F.);
#80820=ORIENTED_EDGE('',*,*,#56979,.T.);
#80821=ORIENTED_EDGE('',*,*,#54114,.F.);
#80822=ORIENTED_EDGE('',*,*,#54110,.T.);
#80823=ORIENTED_EDGE('',*,*,#56980,.F.);
#80824=ORIENTED_EDGE('',*,*,#55122,.F.);
#80825=ORIENTED_EDGE('',*,*,#56981,.F.);
#80826=ORIENTED_EDGE('',*,*,#54066,.F.);
#80827=ORIENTED_EDGE('',*,*,#56981,.T.);
#80828=ORIENTED_EDGE('',*,*,#55121,.F.);
#80829=ORIENTED_EDGE('',*,*,#56982,.F.);
#80830=ORIENTED_EDGE('',*,*,#54075,.F.);
#80831=ORIENTED_EDGE('',*,*,#54065,.T.);
#80832=ORIENTED_EDGE('',*,*,#54069,.F.);
#80833=ORIENTED_EDGE('',*,*,#56983,.F.);
#80834=ORIENTED_EDGE('',*,*,#55123,.F.);
#80835=ORIENTED_EDGE('',*,*,#56980,.T.);
#80836=ORIENTED_EDGE('',*,*,#56982,.T.);
#80837=ORIENTED_EDGE('',*,*,#55120,.F.);
#80838=ORIENTED_EDGE('',*,*,#56984,.F.);
#80839=ORIENTED_EDGE('',*,*,#54060,.F.);
#80840=ORIENTED_EDGE('',*,*,#56983,.T.);
#80841=ORIENTED_EDGE('',*,*,#54073,.F.);
#80842=ORIENTED_EDGE('',*,*,#56985,.F.);
#80843=ORIENTED_EDGE('',*,*,#55112,.F.);
#80844=ORIENTED_EDGE('',*,*,#56984,.T.);
#80845=ORIENTED_EDGE('',*,*,#55119,.F.);
#80846=ORIENTED_EDGE('',*,*,#56986,.F.);
#80847=ORIENTED_EDGE('',*,*,#54077,.F.);
#80848=ORIENTED_EDGE('',*,*,#56985,.T.);
#80849=ORIENTED_EDGE('',*,*,#52168,.F.);
#80850=ORIENTED_EDGE('',*,*,#56987,.F.);
#80851=ORIENTED_EDGE('',*,*,#55113,.F.);
#80852=ORIENTED_EDGE('',*,*,#56986,.T.);
#80853=ORIENTED_EDGE('',*,*,#55118,.F.);
#80854=ORIENTED_EDGE('',*,*,#56988,.F.);
#80855=ORIENTED_EDGE('',*,*,#54052,.T.);
#80856=ORIENTED_EDGE('',*,*,#54056,.F.);
#80857=ORIENTED_EDGE('',*,*,#56987,.T.);
#80858=ORIENTED_EDGE('',*,*,#52167,.F.);
#80859=ORIENTED_EDGE('',*,*,#56989,.F.);
#80860=ORIENTED_EDGE('',*,*,#56360,.F.);
#80861=ORIENTED_EDGE('',*,*,#56988,.T.);
#80862=ORIENTED_EDGE('',*,*,#55117,.F.);
#80863=ORIENTED_EDGE('',*,*,#56990,.F.);
#80864=ORIENTED_EDGE('',*,*,#54053,.F.);
#80865=ORIENTED_EDGE('',*,*,#56989,.T.);
#80866=ORIENTED_EDGE('',*,*,#52166,.F.);
#80867=ORIENTED_EDGE('',*,*,#56991,.F.);
#80868=ORIENTED_EDGE('',*,*,#55097,.F.);
#80869=ORIENTED_EDGE('',*,*,#56990,.T.);
#80870=ORIENTED_EDGE('',*,*,#55116,.F.);
#80871=ORIENTED_EDGE('',*,*,#56992,.F.);
#80872=ORIENTED_EDGE('',*,*,#54071,.F.);
#80873=ORIENTED_EDGE('',*,*,#56991,.T.);
#80874=ORIENTED_EDGE('',*,*,#52165,.F.);
#80875=ORIENTED_EDGE('',*,*,#56993,.F.);
#80876=ORIENTED_EDGE('',*,*,#56362,.F.);
#80877=ORIENTED_EDGE('',*,*,#56992,.T.);
#80878=ORIENTED_EDGE('',*,*,#55115,.F.);
#80879=ORIENTED_EDGE('',*,*,#56994,.F.);
#80880=ORIENTED_EDGE('',*,*,#52498,.F.);
#80881=ORIENTED_EDGE('',*,*,#56993,.T.);
#80882=ORIENTED_EDGE('',*,*,#52164,.F.);
#80883=ORIENTED_EDGE('',*,*,#56995,.F.);
#80884=ORIENTED_EDGE('',*,*,#55103,.F.);
#80885=ORIENTED_EDGE('',*,*,#56994,.T.);
#80886=ORIENTED_EDGE('',*,*,#56361,.F.);
#80887=ORIENTED_EDGE('',*,*,#56996,.F.);
#80888=ORIENTED_EDGE('',*,*,#52499,.F.);
#80889=ORIENTED_EDGE('',*,*,#56995,.T.);
#80890=ORIENTED_EDGE('',*,*,#54102,.F.);
#80891=ORIENTED_EDGE('',*,*,#56997,.F.);
#80892=ORIENTED_EDGE('',*,*,#55104,.F.);
#80893=ORIENTED_EDGE('',*,*,#56996,.T.);
#80894=ORIENTED_EDGE('',*,*,#55099,.F.);
#80895=ORIENTED_EDGE('',*,*,#56998,.F.);
#80896=ORIENTED_EDGE('',*,*,#52500,.F.);
#80897=ORIENTED_EDGE('',*,*,#54097,.F.);
#80898=ORIENTED_EDGE('',*,*,#54093,.T.);
#80899=ORIENTED_EDGE('',*,*,#56999,.F.);
#80900=ORIENTED_EDGE('',*,*,#55105,.F.);
#80901=ORIENTED_EDGE('',*,*,#56997,.T.);
#80902=ORIENTED_EDGE('',*,*,#56998,.T.);
#80903=ORIENTED_EDGE('',*,*,#56363,.F.);
#80904=ORIENTED_EDGE('',*,*,#57000,.F.);
#80905=ORIENTED_EDGE('',*,*,#52501,.F.);
#80906=ORIENTED_EDGE('',*,*,#56999,.T.);
#80907=ORIENTED_EDGE('',*,*,#54092,.F.);
#80908=ORIENTED_EDGE('',*,*,#57001,.F.);
#80909=ORIENTED_EDGE('',*,*,#55106,.F.);
#80910=ORIENTED_EDGE('',*,*,#57000,.T.);
#80911=ORIENTED_EDGE('',*,*,#55101,.F.);
#80912=ORIENTED_EDGE('',*,*,#57002,.F.);
#80913=ORIENTED_EDGE('',*,*,#52502,.F.);
#80914=ORIENTED_EDGE('',*,*,#57001,.T.);
#80915=ORIENTED_EDGE('',*,*,#54104,.F.);
#80916=ORIENTED_EDGE('',*,*,#57003,.F.);
#80917=ORIENTED_EDGE('',*,*,#55107,.F.);
#80918=ORIENTED_EDGE('',*,*,#57002,.T.);
#80919=ORIENTED_EDGE('',*,*,#55100,.F.);
#80920=ORIENTED_EDGE('',*,*,#57004,.F.);
#80921=ORIENTED_EDGE('',*,*,#54100,.F.);
#80922=ORIENTED_EDGE('',*,*,#57003,.T.);
#80923=ORIENTED_EDGE('',*,*,#54088,.F.);
#80924=ORIENTED_EDGE('',*,*,#57005,.F.);
#80925=ORIENTED_EDGE('',*,*,#55108,.F.);
#80926=ORIENTED_EDGE('',*,*,#57004,.T.);
#80927=ORIENTED_EDGE('',*,*,#55111,.F.);
#80928=ORIENTED_EDGE('',*,*,#57006,.F.);
#80929=ORIENTED_EDGE('',*,*,#54079,.F.);
#80930=ORIENTED_EDGE('',*,*,#57005,.T.);
#80931=ORIENTED_EDGE('',*,*,#54106,.F.);
#80932=ORIENTED_EDGE('',*,*,#57007,.F.);
#80933=ORIENTED_EDGE('',*,*,#55109,.F.);
#80934=ORIENTED_EDGE('',*,*,#57006,.T.);
#80935=ORIENTED_EDGE('',*,*,#55110,.F.);
#80936=ORIENTED_EDGE('',*,*,#57007,.T.);
#80937=ORIENTED_EDGE('',*,*,#54084,.F.);
#80938=ORIENTED_EDGE('',*,*,#54080,.T.);
#80939=ORIENTED_EDGE('',*,*,#57008,.F.);
#80940=ORIENTED_EDGE('',*,*,#55150,.F.);
#80941=ORIENTED_EDGE('',*,*,#57009,.F.);
#80942=ORIENTED_EDGE('',*,*,#54036,.F.);
#80943=ORIENTED_EDGE('',*,*,#57009,.T.);
#80944=ORIENTED_EDGE('',*,*,#55149,.F.);
#80945=ORIENTED_EDGE('',*,*,#57010,.F.);
#80946=ORIENTED_EDGE('',*,*,#54045,.F.);
#80947=ORIENTED_EDGE('',*,*,#54035,.T.);
#80948=ORIENTED_EDGE('',*,*,#54039,.F.);
#80949=ORIENTED_EDGE('',*,*,#57011,.F.);
#80950=ORIENTED_EDGE('',*,*,#55151,.F.);
#80951=ORIENTED_EDGE('',*,*,#57008,.T.);
#80952=ORIENTED_EDGE('',*,*,#57010,.T.);
#80953=ORIENTED_EDGE('',*,*,#55148,.F.);
#80954=ORIENTED_EDGE('',*,*,#57012,.F.);
#80955=ORIENTED_EDGE('',*,*,#54030,.F.);
#80956=ORIENTED_EDGE('',*,*,#57011,.T.);
#80957=ORIENTED_EDGE('',*,*,#54043,.F.);
#80958=ORIENTED_EDGE('',*,*,#57013,.F.);
#80959=ORIENTED_EDGE('',*,*,#55140,.F.);
#80960=ORIENTED_EDGE('',*,*,#57012,.T.);
#80961=ORIENTED_EDGE('',*,*,#55147,.F.);
#80962=ORIENTED_EDGE('',*,*,#57014,.F.);
#80963=ORIENTED_EDGE('',*,*,#54047,.F.);
#80964=ORIENTED_EDGE('',*,*,#57013,.T.);
#80965=ORIENTED_EDGE('',*,*,#52174,.F.);
#80966=ORIENTED_EDGE('',*,*,#57015,.F.);
#80967=ORIENTED_EDGE('',*,*,#55141,.F.);
#80968=ORIENTED_EDGE('',*,*,#57014,.T.);
#80969=ORIENTED_EDGE('',*,*,#55146,.F.);
#80970=ORIENTED_EDGE('',*,*,#57016,.F.);
#80971=ORIENTED_EDGE('',*,*,#54022,.T.);
#80972=ORIENTED_EDGE('',*,*,#54026,.F.);
#80973=ORIENTED_EDGE('',*,*,#57015,.T.);
#80974=ORIENTED_EDGE('',*,*,#52173,.F.);
#80975=ORIENTED_EDGE('',*,*,#57017,.F.);
#80976=ORIENTED_EDGE('',*,*,#56364,.F.);
#80977=ORIENTED_EDGE('',*,*,#57016,.T.);
#80978=ORIENTED_EDGE('',*,*,#55145,.F.);
#80979=ORIENTED_EDGE('',*,*,#57018,.F.);
#80980=ORIENTED_EDGE('',*,*,#54023,.F.);
#80981=ORIENTED_EDGE('',*,*,#57017,.T.);
#80982=ORIENTED_EDGE('',*,*,#52172,.F.);
#80983=ORIENTED_EDGE('',*,*,#57019,.F.);
#80984=ORIENTED_EDGE('',*,*,#55125,.F.);
#80985=ORIENTED_EDGE('',*,*,#57018,.T.);
#80986=ORIENTED_EDGE('',*,*,#55144,.F.);
#80987=ORIENTED_EDGE('',*,*,#57020,.F.);
#80988=ORIENTED_EDGE('',*,*,#54041,.F.);
#80989=ORIENTED_EDGE('',*,*,#57019,.T.);
#80990=ORIENTED_EDGE('',*,*,#52171,.F.);
#80991=ORIENTED_EDGE('',*,*,#57021,.F.);
#80992=ORIENTED_EDGE('',*,*,#56366,.F.);
#80993=ORIENTED_EDGE('',*,*,#57020,.T.);
#80994=ORIENTED_EDGE('',*,*,#55143,.F.);
#80995=ORIENTED_EDGE('',*,*,#57022,.F.);
#80996=ORIENTED_EDGE('',*,*,#52492,.F.);
#80997=ORIENTED_EDGE('',*,*,#57021,.T.);
#80998=ORIENTED_EDGE('',*,*,#52170,.F.);
#80999=ORIENTED_EDGE('',*,*,#57023,.F.);
#81000=ORIENTED_EDGE('',*,*,#55131,.F.);
#81001=ORIENTED_EDGE('',*,*,#57022,.T.);
#81002=ORIENTED_EDGE('',*,*,#56365,.F.);
#81003=ORIENTED_EDGE('',*,*,#57024,.F.);
#81004=ORIENTED_EDGE('',*,*,#52493,.F.);
#81005=ORIENTED_EDGE('',*,*,#57023,.T.);
#81006=ORIENTED_EDGE('',*,*,#54072,.F.);
#81007=ORIENTED_EDGE('',*,*,#57025,.F.);
#81008=ORIENTED_EDGE('',*,*,#55132,.F.);
#81009=ORIENTED_EDGE('',*,*,#57024,.T.);
#81010=ORIENTED_EDGE('',*,*,#55127,.F.);
#81011=ORIENTED_EDGE('',*,*,#57026,.F.);
#81012=ORIENTED_EDGE('',*,*,#52494,.F.);
#81013=ORIENTED_EDGE('',*,*,#54067,.F.);
#81014=ORIENTED_EDGE('',*,*,#54063,.T.);
#81015=ORIENTED_EDGE('',*,*,#57027,.F.);
#81016=ORIENTED_EDGE('',*,*,#55133,.F.);
#81017=ORIENTED_EDGE('',*,*,#57025,.T.);
#81018=ORIENTED_EDGE('',*,*,#57026,.T.);
#81019=ORIENTED_EDGE('',*,*,#56367,.F.);
#81020=ORIENTED_EDGE('',*,*,#57028,.F.);
#81021=ORIENTED_EDGE('',*,*,#52495,.F.);
#81022=ORIENTED_EDGE('',*,*,#57027,.T.);
#81023=ORIENTED_EDGE('',*,*,#54062,.F.);
#81024=ORIENTED_EDGE('',*,*,#57029,.F.);
#81025=ORIENTED_EDGE('',*,*,#55134,.F.);
#81026=ORIENTED_EDGE('',*,*,#57028,.T.);
#81027=ORIENTED_EDGE('',*,*,#55129,.F.);
#81028=ORIENTED_EDGE('',*,*,#57030,.F.);
#81029=ORIENTED_EDGE('',*,*,#52496,.F.);
#81030=ORIENTED_EDGE('',*,*,#57029,.T.);
#81031=ORIENTED_EDGE('',*,*,#54074,.F.);
#81032=ORIENTED_EDGE('',*,*,#57031,.F.);
#81033=ORIENTED_EDGE('',*,*,#55135,.F.);
#81034=ORIENTED_EDGE('',*,*,#57030,.T.);
#81035=ORIENTED_EDGE('',*,*,#55128,.F.);
#81036=ORIENTED_EDGE('',*,*,#57032,.F.);
#81037=ORIENTED_EDGE('',*,*,#54070,.F.);
#81038=ORIENTED_EDGE('',*,*,#57031,.T.);
#81039=ORIENTED_EDGE('',*,*,#54058,.F.);
#81040=ORIENTED_EDGE('',*,*,#57033,.F.);
#81041=ORIENTED_EDGE('',*,*,#55136,.F.);
#81042=ORIENTED_EDGE('',*,*,#57032,.T.);
#81043=ORIENTED_EDGE('',*,*,#55139,.F.);
#81044=ORIENTED_EDGE('',*,*,#57034,.F.);
#81045=ORIENTED_EDGE('',*,*,#54049,.F.);
#81046=ORIENTED_EDGE('',*,*,#57033,.T.);
#81047=ORIENTED_EDGE('',*,*,#54076,.F.);
#81048=ORIENTED_EDGE('',*,*,#57035,.F.);
#81049=ORIENTED_EDGE('',*,*,#55137,.F.);
#81050=ORIENTED_EDGE('',*,*,#57034,.T.);
#81051=ORIENTED_EDGE('',*,*,#55138,.F.);
#81052=ORIENTED_EDGE('',*,*,#57035,.T.);
#81053=ORIENTED_EDGE('',*,*,#54054,.F.);
#81054=ORIENTED_EDGE('',*,*,#54050,.T.);
#81055=ORIENTED_EDGE('',*,*,#57036,.F.);
#81056=ORIENTED_EDGE('',*,*,#55178,.F.);
#81057=ORIENTED_EDGE('',*,*,#57037,.F.);
#81058=ORIENTED_EDGE('',*,*,#54006,.F.);
#81059=ORIENTED_EDGE('',*,*,#57037,.T.);
#81060=ORIENTED_EDGE('',*,*,#55177,.F.);
#81061=ORIENTED_EDGE('',*,*,#57038,.F.);
#81062=ORIENTED_EDGE('',*,*,#54015,.F.);
#81063=ORIENTED_EDGE('',*,*,#54005,.T.);
#81064=ORIENTED_EDGE('',*,*,#54009,.F.);
#81065=ORIENTED_EDGE('',*,*,#57039,.F.);
#81066=ORIENTED_EDGE('',*,*,#55179,.F.);
#81067=ORIENTED_EDGE('',*,*,#57036,.T.);
#81068=ORIENTED_EDGE('',*,*,#57038,.T.);
#81069=ORIENTED_EDGE('',*,*,#55176,.F.);
#81070=ORIENTED_EDGE('',*,*,#57040,.F.);
#81071=ORIENTED_EDGE('',*,*,#54000,.F.);
#81072=ORIENTED_EDGE('',*,*,#57039,.T.);
#81073=ORIENTED_EDGE('',*,*,#54013,.F.);
#81074=ORIENTED_EDGE('',*,*,#57041,.F.);
#81075=ORIENTED_EDGE('',*,*,#55168,.F.);
#81076=ORIENTED_EDGE('',*,*,#57040,.T.);
#81077=ORIENTED_EDGE('',*,*,#55175,.F.);
#81078=ORIENTED_EDGE('',*,*,#57042,.F.);
#81079=ORIENTED_EDGE('',*,*,#54017,.F.);
#81080=ORIENTED_EDGE('',*,*,#57041,.T.);
#81081=ORIENTED_EDGE('',*,*,#52180,.F.);
#81082=ORIENTED_EDGE('',*,*,#57043,.F.);
#81083=ORIENTED_EDGE('',*,*,#55169,.F.);
#81084=ORIENTED_EDGE('',*,*,#57042,.T.);
#81085=ORIENTED_EDGE('',*,*,#55174,.F.);
#81086=ORIENTED_EDGE('',*,*,#57044,.F.);
#81087=ORIENTED_EDGE('',*,*,#53992,.T.);
#81088=ORIENTED_EDGE('',*,*,#53996,.F.);
#81089=ORIENTED_EDGE('',*,*,#57043,.T.);
#81090=ORIENTED_EDGE('',*,*,#52179,.F.);
#81091=ORIENTED_EDGE('',*,*,#57045,.F.);
#81092=ORIENTED_EDGE('',*,*,#56368,.F.);
#81093=ORIENTED_EDGE('',*,*,#57044,.T.);
#81094=ORIENTED_EDGE('',*,*,#55173,.F.);
#81095=ORIENTED_EDGE('',*,*,#57046,.F.);
#81096=ORIENTED_EDGE('',*,*,#53993,.F.);
#81097=ORIENTED_EDGE('',*,*,#57045,.T.);
#81098=ORIENTED_EDGE('',*,*,#52178,.F.);
#81099=ORIENTED_EDGE('',*,*,#57047,.F.);
#81100=ORIENTED_EDGE('',*,*,#55153,.F.);
#81101=ORIENTED_EDGE('',*,*,#57046,.T.);
#81102=ORIENTED_EDGE('',*,*,#55172,.F.);
#81103=ORIENTED_EDGE('',*,*,#57048,.F.);
#81104=ORIENTED_EDGE('',*,*,#54011,.F.);
#81105=ORIENTED_EDGE('',*,*,#57047,.T.);
#81106=ORIENTED_EDGE('',*,*,#52177,.F.);
#81107=ORIENTED_EDGE('',*,*,#57049,.F.);
#81108=ORIENTED_EDGE('',*,*,#56370,.F.);
#81109=ORIENTED_EDGE('',*,*,#57048,.T.);
#81110=ORIENTED_EDGE('',*,*,#55171,.F.);
#81111=ORIENTED_EDGE('',*,*,#57050,.F.);
#81112=ORIENTED_EDGE('',*,*,#52486,.F.);
#81113=ORIENTED_EDGE('',*,*,#57049,.T.);
#81114=ORIENTED_EDGE('',*,*,#52176,.F.);
#81115=ORIENTED_EDGE('',*,*,#57051,.F.);
#81116=ORIENTED_EDGE('',*,*,#55159,.F.);
#81117=ORIENTED_EDGE('',*,*,#57050,.T.);
#81118=ORIENTED_EDGE('',*,*,#56369,.F.);
#81119=ORIENTED_EDGE('',*,*,#57052,.F.);
#81120=ORIENTED_EDGE('',*,*,#52487,.F.);
#81121=ORIENTED_EDGE('',*,*,#57051,.T.);
#81122=ORIENTED_EDGE('',*,*,#54042,.F.);
#81123=ORIENTED_EDGE('',*,*,#57053,.F.);
#81124=ORIENTED_EDGE('',*,*,#55160,.F.);
#81125=ORIENTED_EDGE('',*,*,#57052,.T.);
#81126=ORIENTED_EDGE('',*,*,#55155,.F.);
#81127=ORIENTED_EDGE('',*,*,#57054,.F.);
#81128=ORIENTED_EDGE('',*,*,#52488,.F.);
#81129=ORIENTED_EDGE('',*,*,#54037,.F.);
#81130=ORIENTED_EDGE('',*,*,#54033,.T.);
#81131=ORIENTED_EDGE('',*,*,#57055,.F.);
#81132=ORIENTED_EDGE('',*,*,#55161,.F.);
#81133=ORIENTED_EDGE('',*,*,#57053,.T.);
#81134=ORIENTED_EDGE('',*,*,#57054,.T.);
#81135=ORIENTED_EDGE('',*,*,#56371,.F.);
#81136=ORIENTED_EDGE('',*,*,#57056,.F.);
#81137=ORIENTED_EDGE('',*,*,#52489,.F.);
#81138=ORIENTED_EDGE('',*,*,#57055,.T.);
#81139=ORIENTED_EDGE('',*,*,#54032,.F.);
#81140=ORIENTED_EDGE('',*,*,#57057,.F.);
#81141=ORIENTED_EDGE('',*,*,#55162,.F.);
#81142=ORIENTED_EDGE('',*,*,#57056,.T.);
#81143=ORIENTED_EDGE('',*,*,#55157,.F.);
#81144=ORIENTED_EDGE('',*,*,#57058,.F.);
#81145=ORIENTED_EDGE('',*,*,#52490,.F.);
#81146=ORIENTED_EDGE('',*,*,#57057,.T.);
#81147=ORIENTED_EDGE('',*,*,#54044,.F.);
#81148=ORIENTED_EDGE('',*,*,#57059,.F.);
#81149=ORIENTED_EDGE('',*,*,#55163,.F.);
#81150=ORIENTED_EDGE('',*,*,#57058,.T.);
#81151=ORIENTED_EDGE('',*,*,#55156,.F.);
#81152=ORIENTED_EDGE('',*,*,#57060,.F.);
#81153=ORIENTED_EDGE('',*,*,#54040,.F.);
#81154=ORIENTED_EDGE('',*,*,#57059,.T.);
#81155=ORIENTED_EDGE('',*,*,#54028,.F.);
#81156=ORIENTED_EDGE('',*,*,#57061,.F.);
#81157=ORIENTED_EDGE('',*,*,#55164,.F.);
#81158=ORIENTED_EDGE('',*,*,#57060,.T.);
#81159=ORIENTED_EDGE('',*,*,#55167,.F.);
#81160=ORIENTED_EDGE('',*,*,#57062,.F.);
#81161=ORIENTED_EDGE('',*,*,#54019,.F.);
#81162=ORIENTED_EDGE('',*,*,#57061,.T.);
#81163=ORIENTED_EDGE('',*,*,#54046,.F.);
#81164=ORIENTED_EDGE('',*,*,#57063,.F.);
#81165=ORIENTED_EDGE('',*,*,#55165,.F.);
#81166=ORIENTED_EDGE('',*,*,#57062,.T.);
#81167=ORIENTED_EDGE('',*,*,#55166,.F.);
#81168=ORIENTED_EDGE('',*,*,#57063,.T.);
#81169=ORIENTED_EDGE('',*,*,#54024,.F.);
#81170=ORIENTED_EDGE('',*,*,#54020,.T.);
#81171=ORIENTED_EDGE('',*,*,#57064,.F.);
#81172=ORIENTED_EDGE('',*,*,#55206,.F.);
#81173=ORIENTED_EDGE('',*,*,#57065,.F.);
#81174=ORIENTED_EDGE('',*,*,#53976,.F.);
#81175=ORIENTED_EDGE('',*,*,#57065,.T.);
#81176=ORIENTED_EDGE('',*,*,#55205,.F.);
#81177=ORIENTED_EDGE('',*,*,#57066,.F.);
#81178=ORIENTED_EDGE('',*,*,#53985,.F.);
#81179=ORIENTED_EDGE('',*,*,#53975,.T.);
#81180=ORIENTED_EDGE('',*,*,#53979,.F.);
#81181=ORIENTED_EDGE('',*,*,#57067,.F.);
#81182=ORIENTED_EDGE('',*,*,#55207,.F.);
#81183=ORIENTED_EDGE('',*,*,#57064,.T.);
#81184=ORIENTED_EDGE('',*,*,#57066,.T.);
#81185=ORIENTED_EDGE('',*,*,#55204,.F.);
#81186=ORIENTED_EDGE('',*,*,#57068,.F.);
#81187=ORIENTED_EDGE('',*,*,#53970,.F.);
#81188=ORIENTED_EDGE('',*,*,#57067,.T.);
#81189=ORIENTED_EDGE('',*,*,#53983,.F.);
#81190=ORIENTED_EDGE('',*,*,#57069,.F.);
#81191=ORIENTED_EDGE('',*,*,#55196,.F.);
#81192=ORIENTED_EDGE('',*,*,#57068,.T.);
#81193=ORIENTED_EDGE('',*,*,#55203,.F.);
#81194=ORIENTED_EDGE('',*,*,#57070,.F.);
#81195=ORIENTED_EDGE('',*,*,#53987,.F.);
#81196=ORIENTED_EDGE('',*,*,#57069,.T.);
#81197=ORIENTED_EDGE('',*,*,#52186,.F.);
#81198=ORIENTED_EDGE('',*,*,#57071,.F.);
#81199=ORIENTED_EDGE('',*,*,#55197,.F.);
#81200=ORIENTED_EDGE('',*,*,#57070,.T.);
#81201=ORIENTED_EDGE('',*,*,#55202,.F.);
#81202=ORIENTED_EDGE('',*,*,#57072,.F.);
#81203=ORIENTED_EDGE('',*,*,#53962,.T.);
#81204=ORIENTED_EDGE('',*,*,#53966,.F.);
#81205=ORIENTED_EDGE('',*,*,#57071,.T.);
#81206=ORIENTED_EDGE('',*,*,#52185,.F.);
#81207=ORIENTED_EDGE('',*,*,#57073,.F.);
#81208=ORIENTED_EDGE('',*,*,#56372,.F.);
#81209=ORIENTED_EDGE('',*,*,#57072,.T.);
#81210=ORIENTED_EDGE('',*,*,#55201,.F.);
#81211=ORIENTED_EDGE('',*,*,#57074,.F.);
#81212=ORIENTED_EDGE('',*,*,#53963,.F.);
#81213=ORIENTED_EDGE('',*,*,#57073,.T.);
#81214=ORIENTED_EDGE('',*,*,#52184,.F.);
#81215=ORIENTED_EDGE('',*,*,#57075,.F.);
#81216=ORIENTED_EDGE('',*,*,#55181,.F.);
#81217=ORIENTED_EDGE('',*,*,#57074,.T.);
#81218=ORIENTED_EDGE('',*,*,#55200,.F.);
#81219=ORIENTED_EDGE('',*,*,#57076,.F.);
#81220=ORIENTED_EDGE('',*,*,#53981,.F.);
#81221=ORIENTED_EDGE('',*,*,#57075,.T.);
#81222=ORIENTED_EDGE('',*,*,#52183,.F.);
#81223=ORIENTED_EDGE('',*,*,#57077,.F.);
#81224=ORIENTED_EDGE('',*,*,#56374,.F.);
#81225=ORIENTED_EDGE('',*,*,#57076,.T.);
#81226=ORIENTED_EDGE('',*,*,#55199,.F.);
#81227=ORIENTED_EDGE('',*,*,#57078,.F.);
#81228=ORIENTED_EDGE('',*,*,#52480,.F.);
#81229=ORIENTED_EDGE('',*,*,#57077,.T.);
#81230=ORIENTED_EDGE('',*,*,#52182,.F.);
#81231=ORIENTED_EDGE('',*,*,#57079,.F.);
#81232=ORIENTED_EDGE('',*,*,#55187,.F.);
#81233=ORIENTED_EDGE('',*,*,#57078,.T.);
#81234=ORIENTED_EDGE('',*,*,#56373,.F.);
#81235=ORIENTED_EDGE('',*,*,#57080,.F.);
#81236=ORIENTED_EDGE('',*,*,#52481,.F.);
#81237=ORIENTED_EDGE('',*,*,#57079,.T.);
#81238=ORIENTED_EDGE('',*,*,#54012,.F.);
#81239=ORIENTED_EDGE('',*,*,#57081,.F.);
#81240=ORIENTED_EDGE('',*,*,#55188,.F.);
#81241=ORIENTED_EDGE('',*,*,#57080,.T.);
#81242=ORIENTED_EDGE('',*,*,#55183,.F.);
#81243=ORIENTED_EDGE('',*,*,#57082,.F.);
#81244=ORIENTED_EDGE('',*,*,#52482,.F.);
#81245=ORIENTED_EDGE('',*,*,#54007,.F.);
#81246=ORIENTED_EDGE('',*,*,#54003,.T.);
#81247=ORIENTED_EDGE('',*,*,#57083,.F.);
#81248=ORIENTED_EDGE('',*,*,#55189,.F.);
#81249=ORIENTED_EDGE('',*,*,#57081,.T.);
#81250=ORIENTED_EDGE('',*,*,#57082,.T.);
#81251=ORIENTED_EDGE('',*,*,#56375,.F.);
#81252=ORIENTED_EDGE('',*,*,#57084,.F.);
#81253=ORIENTED_EDGE('',*,*,#52483,.F.);
#81254=ORIENTED_EDGE('',*,*,#57083,.T.);
#81255=ORIENTED_EDGE('',*,*,#54002,.F.);
#81256=ORIENTED_EDGE('',*,*,#57085,.F.);
#81257=ORIENTED_EDGE('',*,*,#55190,.F.);
#81258=ORIENTED_EDGE('',*,*,#57084,.T.);
#81259=ORIENTED_EDGE('',*,*,#55185,.F.);
#81260=ORIENTED_EDGE('',*,*,#57086,.F.);
#81261=ORIENTED_EDGE('',*,*,#52484,.F.);
#81262=ORIENTED_EDGE('',*,*,#57085,.T.);
#81263=ORIENTED_EDGE('',*,*,#54014,.F.);
#81264=ORIENTED_EDGE('',*,*,#57087,.F.);
#81265=ORIENTED_EDGE('',*,*,#55191,.F.);
#81266=ORIENTED_EDGE('',*,*,#57086,.T.);
#81267=ORIENTED_EDGE('',*,*,#55184,.F.);
#81268=ORIENTED_EDGE('',*,*,#57088,.F.);
#81269=ORIENTED_EDGE('',*,*,#54010,.F.);
#81270=ORIENTED_EDGE('',*,*,#57087,.T.);
#81271=ORIENTED_EDGE('',*,*,#53998,.F.);
#81272=ORIENTED_EDGE('',*,*,#57089,.F.);
#81273=ORIENTED_EDGE('',*,*,#55192,.F.);
#81274=ORIENTED_EDGE('',*,*,#57088,.T.);
#81275=ORIENTED_EDGE('',*,*,#55195,.F.);
#81276=ORIENTED_EDGE('',*,*,#57090,.F.);
#81277=ORIENTED_EDGE('',*,*,#53989,.F.);
#81278=ORIENTED_EDGE('',*,*,#57089,.T.);
#81279=ORIENTED_EDGE('',*,*,#54016,.F.);
#81280=ORIENTED_EDGE('',*,*,#57091,.F.);
#81281=ORIENTED_EDGE('',*,*,#55193,.F.);
#81282=ORIENTED_EDGE('',*,*,#57090,.T.);
#81283=ORIENTED_EDGE('',*,*,#55194,.F.);
#81284=ORIENTED_EDGE('',*,*,#57091,.T.);
#81285=ORIENTED_EDGE('',*,*,#53994,.F.);
#81286=ORIENTED_EDGE('',*,*,#53990,.T.);
#81287=ORIENTED_EDGE('',*,*,#57092,.F.);
#81288=ORIENTED_EDGE('',*,*,#55234,.F.);
#81289=ORIENTED_EDGE('',*,*,#57093,.F.);
#81290=ORIENTED_EDGE('',*,*,#53946,.F.);
#81291=ORIENTED_EDGE('',*,*,#57093,.T.);
#81292=ORIENTED_EDGE('',*,*,#55233,.F.);
#81293=ORIENTED_EDGE('',*,*,#57094,.F.);
#81294=ORIENTED_EDGE('',*,*,#53955,.F.);
#81295=ORIENTED_EDGE('',*,*,#53945,.T.);
#81296=ORIENTED_EDGE('',*,*,#53949,.F.);
#81297=ORIENTED_EDGE('',*,*,#57095,.F.);
#81298=ORIENTED_EDGE('',*,*,#55235,.F.);
#81299=ORIENTED_EDGE('',*,*,#57092,.T.);
#81300=ORIENTED_EDGE('',*,*,#57094,.T.);
#81301=ORIENTED_EDGE('',*,*,#55232,.F.);
#81302=ORIENTED_EDGE('',*,*,#57096,.F.);
#81303=ORIENTED_EDGE('',*,*,#53940,.F.);
#81304=ORIENTED_EDGE('',*,*,#57095,.T.);
#81305=ORIENTED_EDGE('',*,*,#53953,.F.);
#81306=ORIENTED_EDGE('',*,*,#57097,.F.);
#81307=ORIENTED_EDGE('',*,*,#55224,.F.);
#81308=ORIENTED_EDGE('',*,*,#57096,.T.);
#81309=ORIENTED_EDGE('',*,*,#55231,.F.);
#81310=ORIENTED_EDGE('',*,*,#57098,.F.);
#81311=ORIENTED_EDGE('',*,*,#53957,.F.);
#81312=ORIENTED_EDGE('',*,*,#57097,.T.);
#81313=ORIENTED_EDGE('',*,*,#52192,.F.);
#81314=ORIENTED_EDGE('',*,*,#57099,.F.);
#81315=ORIENTED_EDGE('',*,*,#55225,.F.);
#81316=ORIENTED_EDGE('',*,*,#57098,.T.);
#81317=ORIENTED_EDGE('',*,*,#55230,.F.);
#81318=ORIENTED_EDGE('',*,*,#57100,.F.);
#81319=ORIENTED_EDGE('',*,*,#53932,.T.);
#81320=ORIENTED_EDGE('',*,*,#53936,.F.);
#81321=ORIENTED_EDGE('',*,*,#57099,.T.);
#81322=ORIENTED_EDGE('',*,*,#52191,.F.);
#81323=ORIENTED_EDGE('',*,*,#57101,.F.);
#81324=ORIENTED_EDGE('',*,*,#56376,.F.);
#81325=ORIENTED_EDGE('',*,*,#57100,.T.);
#81326=ORIENTED_EDGE('',*,*,#55229,.F.);
#81327=ORIENTED_EDGE('',*,*,#57102,.F.);
#81328=ORIENTED_EDGE('',*,*,#53933,.F.);
#81329=ORIENTED_EDGE('',*,*,#57101,.T.);
#81330=ORIENTED_EDGE('',*,*,#52190,.F.);
#81331=ORIENTED_EDGE('',*,*,#57103,.F.);
#81332=ORIENTED_EDGE('',*,*,#55209,.F.);
#81333=ORIENTED_EDGE('',*,*,#57102,.T.);
#81334=ORIENTED_EDGE('',*,*,#55228,.F.);
#81335=ORIENTED_EDGE('',*,*,#57104,.F.);
#81336=ORIENTED_EDGE('',*,*,#53951,.F.);
#81337=ORIENTED_EDGE('',*,*,#57103,.T.);
#81338=ORIENTED_EDGE('',*,*,#52189,.F.);
#81339=ORIENTED_EDGE('',*,*,#57105,.F.);
#81340=ORIENTED_EDGE('',*,*,#56378,.F.);
#81341=ORIENTED_EDGE('',*,*,#57104,.T.);
#81342=ORIENTED_EDGE('',*,*,#55227,.F.);
#81343=ORIENTED_EDGE('',*,*,#57106,.F.);
#81344=ORIENTED_EDGE('',*,*,#52474,.F.);
#81345=ORIENTED_EDGE('',*,*,#57105,.T.);
#81346=ORIENTED_EDGE('',*,*,#52188,.F.);
#81347=ORIENTED_EDGE('',*,*,#57107,.F.);
#81348=ORIENTED_EDGE('',*,*,#55215,.F.);
#81349=ORIENTED_EDGE('',*,*,#57106,.T.);
#81350=ORIENTED_EDGE('',*,*,#56377,.F.);
#81351=ORIENTED_EDGE('',*,*,#57108,.F.);
#81352=ORIENTED_EDGE('',*,*,#52475,.F.);
#81353=ORIENTED_EDGE('',*,*,#57107,.T.);
#81354=ORIENTED_EDGE('',*,*,#53982,.F.);
#81355=ORIENTED_EDGE('',*,*,#57109,.F.);
#81356=ORIENTED_EDGE('',*,*,#55216,.F.);
#81357=ORIENTED_EDGE('',*,*,#57108,.T.);
#81358=ORIENTED_EDGE('',*,*,#55211,.F.);
#81359=ORIENTED_EDGE('',*,*,#57110,.F.);
#81360=ORIENTED_EDGE('',*,*,#52476,.F.);
#81361=ORIENTED_EDGE('',*,*,#53977,.F.);
#81362=ORIENTED_EDGE('',*,*,#53973,.T.);
#81363=ORIENTED_EDGE('',*,*,#57111,.F.);
#81364=ORIENTED_EDGE('',*,*,#55217,.F.);
#81365=ORIENTED_EDGE('',*,*,#57109,.T.);
#81366=ORIENTED_EDGE('',*,*,#57110,.T.);
#81367=ORIENTED_EDGE('',*,*,#56379,.F.);
#81368=ORIENTED_EDGE('',*,*,#57112,.F.);
#81369=ORIENTED_EDGE('',*,*,#52477,.F.);
#81370=ORIENTED_EDGE('',*,*,#57111,.T.);
#81371=ORIENTED_EDGE('',*,*,#53972,.F.);
#81372=ORIENTED_EDGE('',*,*,#57113,.F.);
#81373=ORIENTED_EDGE('',*,*,#55218,.F.);
#81374=ORIENTED_EDGE('',*,*,#57112,.T.);
#81375=ORIENTED_EDGE('',*,*,#55213,.F.);
#81376=ORIENTED_EDGE('',*,*,#57114,.F.);
#81377=ORIENTED_EDGE('',*,*,#52478,.F.);
#81378=ORIENTED_EDGE('',*,*,#57113,.T.);
#81379=ORIENTED_EDGE('',*,*,#53984,.F.);
#81380=ORIENTED_EDGE('',*,*,#57115,.F.);
#81381=ORIENTED_EDGE('',*,*,#55219,.F.);
#81382=ORIENTED_EDGE('',*,*,#57114,.T.);
#81383=ORIENTED_EDGE('',*,*,#55212,.F.);
#81384=ORIENTED_EDGE('',*,*,#57116,.F.);
#81385=ORIENTED_EDGE('',*,*,#53980,.F.);
#81386=ORIENTED_EDGE('',*,*,#57115,.T.);
#81387=ORIENTED_EDGE('',*,*,#53968,.F.);
#81388=ORIENTED_EDGE('',*,*,#57117,.F.);
#81389=ORIENTED_EDGE('',*,*,#55220,.F.);
#81390=ORIENTED_EDGE('',*,*,#57116,.T.);
#81391=ORIENTED_EDGE('',*,*,#55223,.F.);
#81392=ORIENTED_EDGE('',*,*,#57118,.F.);
#81393=ORIENTED_EDGE('',*,*,#53959,.F.);
#81394=ORIENTED_EDGE('',*,*,#57117,.T.);
#81395=ORIENTED_EDGE('',*,*,#53986,.F.);
#81396=ORIENTED_EDGE('',*,*,#57119,.F.);
#81397=ORIENTED_EDGE('',*,*,#55221,.F.);
#81398=ORIENTED_EDGE('',*,*,#57118,.T.);
#81399=ORIENTED_EDGE('',*,*,#55222,.F.);
#81400=ORIENTED_EDGE('',*,*,#57119,.T.);
#81401=ORIENTED_EDGE('',*,*,#53964,.F.);
#81402=ORIENTED_EDGE('',*,*,#53960,.T.);
#81403=ORIENTED_EDGE('',*,*,#57120,.F.);
#81404=ORIENTED_EDGE('',*,*,#55262,.F.);
#81405=ORIENTED_EDGE('',*,*,#57121,.F.);
#81406=ORIENTED_EDGE('',*,*,#53916,.F.);
#81407=ORIENTED_EDGE('',*,*,#57121,.T.);
#81408=ORIENTED_EDGE('',*,*,#55261,.F.);
#81409=ORIENTED_EDGE('',*,*,#57122,.F.);
#81410=ORIENTED_EDGE('',*,*,#53925,.F.);
#81411=ORIENTED_EDGE('',*,*,#53915,.T.);
#81412=ORIENTED_EDGE('',*,*,#53919,.F.);
#81413=ORIENTED_EDGE('',*,*,#57123,.F.);
#81414=ORIENTED_EDGE('',*,*,#55263,.F.);
#81415=ORIENTED_EDGE('',*,*,#57120,.T.);
#81416=ORIENTED_EDGE('',*,*,#57122,.T.);
#81417=ORIENTED_EDGE('',*,*,#55260,.F.);
#81418=ORIENTED_EDGE('',*,*,#57124,.F.);
#81419=ORIENTED_EDGE('',*,*,#53910,.F.);
#81420=ORIENTED_EDGE('',*,*,#57123,.T.);
#81421=ORIENTED_EDGE('',*,*,#53923,.F.);
#81422=ORIENTED_EDGE('',*,*,#57125,.F.);
#81423=ORIENTED_EDGE('',*,*,#55252,.F.);
#81424=ORIENTED_EDGE('',*,*,#57124,.T.);
#81425=ORIENTED_EDGE('',*,*,#55259,.F.);
#81426=ORIENTED_EDGE('',*,*,#57126,.F.);
#81427=ORIENTED_EDGE('',*,*,#53927,.F.);
#81428=ORIENTED_EDGE('',*,*,#57125,.T.);
#81429=ORIENTED_EDGE('',*,*,#52198,.F.);
#81430=ORIENTED_EDGE('',*,*,#57127,.F.);
#81431=ORIENTED_EDGE('',*,*,#55253,.F.);
#81432=ORIENTED_EDGE('',*,*,#57126,.T.);
#81433=ORIENTED_EDGE('',*,*,#55258,.F.);
#81434=ORIENTED_EDGE('',*,*,#57128,.F.);
#81435=ORIENTED_EDGE('',*,*,#53902,.T.);
#81436=ORIENTED_EDGE('',*,*,#53906,.F.);
#81437=ORIENTED_EDGE('',*,*,#57127,.T.);
#81438=ORIENTED_EDGE('',*,*,#52197,.F.);
#81439=ORIENTED_EDGE('',*,*,#57129,.F.);
#81440=ORIENTED_EDGE('',*,*,#56380,.F.);
#81441=ORIENTED_EDGE('',*,*,#57128,.T.);
#81442=ORIENTED_EDGE('',*,*,#55257,.F.);
#81443=ORIENTED_EDGE('',*,*,#57130,.F.);
#81444=ORIENTED_EDGE('',*,*,#53903,.F.);
#81445=ORIENTED_EDGE('',*,*,#57129,.T.);
#81446=ORIENTED_EDGE('',*,*,#52196,.F.);
#81447=ORIENTED_EDGE('',*,*,#57131,.F.);
#81448=ORIENTED_EDGE('',*,*,#55237,.F.);
#81449=ORIENTED_EDGE('',*,*,#57130,.T.);
#81450=ORIENTED_EDGE('',*,*,#55256,.F.);
#81451=ORIENTED_EDGE('',*,*,#57132,.F.);
#81452=ORIENTED_EDGE('',*,*,#53921,.F.);
#81453=ORIENTED_EDGE('',*,*,#57131,.T.);
#81454=ORIENTED_EDGE('',*,*,#52195,.F.);
#81455=ORIENTED_EDGE('',*,*,#57133,.F.);
#81456=ORIENTED_EDGE('',*,*,#56382,.F.);
#81457=ORIENTED_EDGE('',*,*,#57132,.T.);
#81458=ORIENTED_EDGE('',*,*,#55255,.F.);
#81459=ORIENTED_EDGE('',*,*,#57134,.F.);
#81460=ORIENTED_EDGE('',*,*,#52468,.F.);
#81461=ORIENTED_EDGE('',*,*,#57133,.T.);
#81462=ORIENTED_EDGE('',*,*,#52194,.F.);
#81463=ORIENTED_EDGE('',*,*,#57135,.F.);
#81464=ORIENTED_EDGE('',*,*,#55243,.F.);
#81465=ORIENTED_EDGE('',*,*,#57134,.T.);
#81466=ORIENTED_EDGE('',*,*,#56381,.F.);
#81467=ORIENTED_EDGE('',*,*,#57136,.F.);
#81468=ORIENTED_EDGE('',*,*,#52469,.F.);
#81469=ORIENTED_EDGE('',*,*,#57135,.T.);
#81470=ORIENTED_EDGE('',*,*,#53952,.F.);
#81471=ORIENTED_EDGE('',*,*,#57137,.F.);
#81472=ORIENTED_EDGE('',*,*,#55244,.F.);
#81473=ORIENTED_EDGE('',*,*,#57136,.T.);
#81474=ORIENTED_EDGE('',*,*,#55239,.F.);
#81475=ORIENTED_EDGE('',*,*,#57138,.F.);
#81476=ORIENTED_EDGE('',*,*,#52470,.F.);
#81477=ORIENTED_EDGE('',*,*,#53947,.F.);
#81478=ORIENTED_EDGE('',*,*,#53943,.T.);
#81479=ORIENTED_EDGE('',*,*,#57139,.F.);
#81480=ORIENTED_EDGE('',*,*,#55245,.F.);
#81481=ORIENTED_EDGE('',*,*,#57137,.T.);
#81482=ORIENTED_EDGE('',*,*,#57138,.T.);
#81483=ORIENTED_EDGE('',*,*,#56383,.F.);
#81484=ORIENTED_EDGE('',*,*,#57140,.F.);
#81485=ORIENTED_EDGE('',*,*,#52471,.F.);
#81486=ORIENTED_EDGE('',*,*,#57139,.T.);
#81487=ORIENTED_EDGE('',*,*,#53942,.F.);
#81488=ORIENTED_EDGE('',*,*,#57141,.F.);
#81489=ORIENTED_EDGE('',*,*,#55246,.F.);
#81490=ORIENTED_EDGE('',*,*,#57140,.T.);
#81491=ORIENTED_EDGE('',*,*,#55241,.F.);
#81492=ORIENTED_EDGE('',*,*,#57142,.F.);
#81493=ORIENTED_EDGE('',*,*,#52472,.F.);
#81494=ORIENTED_EDGE('',*,*,#57141,.T.);
#81495=ORIENTED_EDGE('',*,*,#53954,.F.);
#81496=ORIENTED_EDGE('',*,*,#57143,.F.);
#81497=ORIENTED_EDGE('',*,*,#55247,.F.);
#81498=ORIENTED_EDGE('',*,*,#57142,.T.);
#81499=ORIENTED_EDGE('',*,*,#55240,.F.);
#81500=ORIENTED_EDGE('',*,*,#57144,.F.);
#81501=ORIENTED_EDGE('',*,*,#53950,.F.);
#81502=ORIENTED_EDGE('',*,*,#57143,.T.);
#81503=ORIENTED_EDGE('',*,*,#53938,.F.);
#81504=ORIENTED_EDGE('',*,*,#57145,.F.);
#81505=ORIENTED_EDGE('',*,*,#55248,.F.);
#81506=ORIENTED_EDGE('',*,*,#57144,.T.);
#81507=ORIENTED_EDGE('',*,*,#55251,.F.);
#81508=ORIENTED_EDGE('',*,*,#57146,.F.);
#81509=ORIENTED_EDGE('',*,*,#53929,.F.);
#81510=ORIENTED_EDGE('',*,*,#57145,.T.);
#81511=ORIENTED_EDGE('',*,*,#53956,.F.);
#81512=ORIENTED_EDGE('',*,*,#57147,.F.);
#81513=ORIENTED_EDGE('',*,*,#55249,.F.);
#81514=ORIENTED_EDGE('',*,*,#57146,.T.);
#81515=ORIENTED_EDGE('',*,*,#55250,.F.);
#81516=ORIENTED_EDGE('',*,*,#57147,.T.);
#81517=ORIENTED_EDGE('',*,*,#53934,.F.);
#81518=ORIENTED_EDGE('',*,*,#53930,.T.);
#81519=ORIENTED_EDGE('',*,*,#57148,.F.);
#81520=ORIENTED_EDGE('',*,*,#55290,.F.);
#81521=ORIENTED_EDGE('',*,*,#57149,.F.);
#81522=ORIENTED_EDGE('',*,*,#53886,.F.);
#81523=ORIENTED_EDGE('',*,*,#57149,.T.);
#81524=ORIENTED_EDGE('',*,*,#55289,.F.);
#81525=ORIENTED_EDGE('',*,*,#57150,.F.);
#81526=ORIENTED_EDGE('',*,*,#53895,.F.);
#81527=ORIENTED_EDGE('',*,*,#53885,.T.);
#81528=ORIENTED_EDGE('',*,*,#53889,.F.);
#81529=ORIENTED_EDGE('',*,*,#57151,.F.);
#81530=ORIENTED_EDGE('',*,*,#55291,.F.);
#81531=ORIENTED_EDGE('',*,*,#57148,.T.);
#81532=ORIENTED_EDGE('',*,*,#57150,.T.);
#81533=ORIENTED_EDGE('',*,*,#55288,.F.);
#81534=ORIENTED_EDGE('',*,*,#57152,.F.);
#81535=ORIENTED_EDGE('',*,*,#53880,.F.);
#81536=ORIENTED_EDGE('',*,*,#57151,.T.);
#81537=ORIENTED_EDGE('',*,*,#53893,.F.);
#81538=ORIENTED_EDGE('',*,*,#57153,.F.);
#81539=ORIENTED_EDGE('',*,*,#55280,.F.);
#81540=ORIENTED_EDGE('',*,*,#57152,.T.);
#81541=ORIENTED_EDGE('',*,*,#55287,.F.);
#81542=ORIENTED_EDGE('',*,*,#57154,.F.);
#81543=ORIENTED_EDGE('',*,*,#53897,.F.);
#81544=ORIENTED_EDGE('',*,*,#57153,.T.);
#81545=ORIENTED_EDGE('',*,*,#52204,.F.);
#81546=ORIENTED_EDGE('',*,*,#57155,.F.);
#81547=ORIENTED_EDGE('',*,*,#55281,.F.);
#81548=ORIENTED_EDGE('',*,*,#57154,.T.);
#81549=ORIENTED_EDGE('',*,*,#55286,.F.);
#81550=ORIENTED_EDGE('',*,*,#57156,.F.);
#81551=ORIENTED_EDGE('',*,*,#53872,.T.);
#81552=ORIENTED_EDGE('',*,*,#53876,.F.);
#81553=ORIENTED_EDGE('',*,*,#57155,.T.);
#81554=ORIENTED_EDGE('',*,*,#52203,.F.);
#81555=ORIENTED_EDGE('',*,*,#57157,.F.);
#81556=ORIENTED_EDGE('',*,*,#56384,.F.);
#81557=ORIENTED_EDGE('',*,*,#57156,.T.);
#81558=ORIENTED_EDGE('',*,*,#55285,.F.);
#81559=ORIENTED_EDGE('',*,*,#57158,.F.);
#81560=ORIENTED_EDGE('',*,*,#53873,.F.);
#81561=ORIENTED_EDGE('',*,*,#57157,.T.);
#81562=ORIENTED_EDGE('',*,*,#52202,.F.);
#81563=ORIENTED_EDGE('',*,*,#57159,.F.);
#81564=ORIENTED_EDGE('',*,*,#55265,.F.);
#81565=ORIENTED_EDGE('',*,*,#57158,.T.);
#81566=ORIENTED_EDGE('',*,*,#55284,.F.);
#81567=ORIENTED_EDGE('',*,*,#57160,.F.);
#81568=ORIENTED_EDGE('',*,*,#53891,.F.);
#81569=ORIENTED_EDGE('',*,*,#57159,.T.);
#81570=ORIENTED_EDGE('',*,*,#52201,.F.);
#81571=ORIENTED_EDGE('',*,*,#57161,.F.);
#81572=ORIENTED_EDGE('',*,*,#56386,.F.);
#81573=ORIENTED_EDGE('',*,*,#57160,.T.);
#81574=ORIENTED_EDGE('',*,*,#55283,.F.);
#81575=ORIENTED_EDGE('',*,*,#57162,.F.);
#81576=ORIENTED_EDGE('',*,*,#52462,.F.);
#81577=ORIENTED_EDGE('',*,*,#57161,.T.);
#81578=ORIENTED_EDGE('',*,*,#52200,.F.);
#81579=ORIENTED_EDGE('',*,*,#57163,.F.);
#81580=ORIENTED_EDGE('',*,*,#55271,.F.);
#81581=ORIENTED_EDGE('',*,*,#57162,.T.);
#81582=ORIENTED_EDGE('',*,*,#56385,.F.);
#81583=ORIENTED_EDGE('',*,*,#57164,.F.);
#81584=ORIENTED_EDGE('',*,*,#52463,.F.);
#81585=ORIENTED_EDGE('',*,*,#57163,.T.);
#81586=ORIENTED_EDGE('',*,*,#53922,.F.);
#81587=ORIENTED_EDGE('',*,*,#57165,.F.);
#81588=ORIENTED_EDGE('',*,*,#55272,.F.);
#81589=ORIENTED_EDGE('',*,*,#57164,.T.);
#81590=ORIENTED_EDGE('',*,*,#55267,.F.);
#81591=ORIENTED_EDGE('',*,*,#57166,.F.);
#81592=ORIENTED_EDGE('',*,*,#52464,.F.);
#81593=ORIENTED_EDGE('',*,*,#53917,.F.);
#81594=ORIENTED_EDGE('',*,*,#53913,.T.);
#81595=ORIENTED_EDGE('',*,*,#57167,.F.);
#81596=ORIENTED_EDGE('',*,*,#55273,.F.);
#81597=ORIENTED_EDGE('',*,*,#57165,.T.);
#81598=ORIENTED_EDGE('',*,*,#57166,.T.);
#81599=ORIENTED_EDGE('',*,*,#56387,.F.);
#81600=ORIENTED_EDGE('',*,*,#57168,.F.);
#81601=ORIENTED_EDGE('',*,*,#52465,.F.);
#81602=ORIENTED_EDGE('',*,*,#57167,.T.);
#81603=ORIENTED_EDGE('',*,*,#53912,.F.);
#81604=ORIENTED_EDGE('',*,*,#57169,.F.);
#81605=ORIENTED_EDGE('',*,*,#55274,.F.);
#81606=ORIENTED_EDGE('',*,*,#57168,.T.);
#81607=ORIENTED_EDGE('',*,*,#55269,.F.);
#81608=ORIENTED_EDGE('',*,*,#57170,.F.);
#81609=ORIENTED_EDGE('',*,*,#52466,.F.);
#81610=ORIENTED_EDGE('',*,*,#57169,.T.);
#81611=ORIENTED_EDGE('',*,*,#53924,.F.);
#81612=ORIENTED_EDGE('',*,*,#57171,.F.);
#81613=ORIENTED_EDGE('',*,*,#55275,.F.);
#81614=ORIENTED_EDGE('',*,*,#57170,.T.);
#81615=ORIENTED_EDGE('',*,*,#55268,.F.);
#81616=ORIENTED_EDGE('',*,*,#57172,.F.);
#81617=ORIENTED_EDGE('',*,*,#53920,.F.);
#81618=ORIENTED_EDGE('',*,*,#57171,.T.);
#81619=ORIENTED_EDGE('',*,*,#53908,.F.);
#81620=ORIENTED_EDGE('',*,*,#57173,.F.);
#81621=ORIENTED_EDGE('',*,*,#55276,.F.);
#81622=ORIENTED_EDGE('',*,*,#57172,.T.);
#81623=ORIENTED_EDGE('',*,*,#55279,.F.);
#81624=ORIENTED_EDGE('',*,*,#57174,.F.);
#81625=ORIENTED_EDGE('',*,*,#53899,.F.);
#81626=ORIENTED_EDGE('',*,*,#57173,.T.);
#81627=ORIENTED_EDGE('',*,*,#53926,.F.);
#81628=ORIENTED_EDGE('',*,*,#57175,.F.);
#81629=ORIENTED_EDGE('',*,*,#55277,.F.);
#81630=ORIENTED_EDGE('',*,*,#57174,.T.);
#81631=ORIENTED_EDGE('',*,*,#55278,.F.);
#81632=ORIENTED_EDGE('',*,*,#57175,.T.);
#81633=ORIENTED_EDGE('',*,*,#53904,.F.);
#81634=ORIENTED_EDGE('',*,*,#53900,.T.);
#81635=ORIENTED_EDGE('',*,*,#57176,.F.);
#81636=ORIENTED_EDGE('',*,*,#55318,.F.);
#81637=ORIENTED_EDGE('',*,*,#57177,.F.);
#81638=ORIENTED_EDGE('',*,*,#53856,.F.);
#81639=ORIENTED_EDGE('',*,*,#57177,.T.);
#81640=ORIENTED_EDGE('',*,*,#55317,.F.);
#81641=ORIENTED_EDGE('',*,*,#57178,.F.);
#81642=ORIENTED_EDGE('',*,*,#53865,.F.);
#81643=ORIENTED_EDGE('',*,*,#53855,.T.);
#81644=ORIENTED_EDGE('',*,*,#53859,.F.);
#81645=ORIENTED_EDGE('',*,*,#57179,.F.);
#81646=ORIENTED_EDGE('',*,*,#55319,.F.);
#81647=ORIENTED_EDGE('',*,*,#57176,.T.);
#81648=ORIENTED_EDGE('',*,*,#57178,.T.);
#81649=ORIENTED_EDGE('',*,*,#55316,.F.);
#81650=ORIENTED_EDGE('',*,*,#57180,.F.);
#81651=ORIENTED_EDGE('',*,*,#53850,.F.);
#81652=ORIENTED_EDGE('',*,*,#57179,.T.);
#81653=ORIENTED_EDGE('',*,*,#53863,.F.);
#81654=ORIENTED_EDGE('',*,*,#57181,.F.);
#81655=ORIENTED_EDGE('',*,*,#55308,.F.);
#81656=ORIENTED_EDGE('',*,*,#57180,.T.);
#81657=ORIENTED_EDGE('',*,*,#55315,.F.);
#81658=ORIENTED_EDGE('',*,*,#57182,.F.);
#81659=ORIENTED_EDGE('',*,*,#53867,.F.);
#81660=ORIENTED_EDGE('',*,*,#57181,.T.);
#81661=ORIENTED_EDGE('',*,*,#52210,.F.);
#81662=ORIENTED_EDGE('',*,*,#57183,.F.);
#81663=ORIENTED_EDGE('',*,*,#55309,.F.);
#81664=ORIENTED_EDGE('',*,*,#57182,.T.);
#81665=ORIENTED_EDGE('',*,*,#55314,.F.);
#81666=ORIENTED_EDGE('',*,*,#57184,.F.);
#81667=ORIENTED_EDGE('',*,*,#53842,.T.);
#81668=ORIENTED_EDGE('',*,*,#53846,.F.);
#81669=ORIENTED_EDGE('',*,*,#57183,.T.);
#81670=ORIENTED_EDGE('',*,*,#52209,.F.);
#81671=ORIENTED_EDGE('',*,*,#57185,.F.);
#81672=ORIENTED_EDGE('',*,*,#56388,.F.);
#81673=ORIENTED_EDGE('',*,*,#57184,.T.);
#81674=ORIENTED_EDGE('',*,*,#55313,.F.);
#81675=ORIENTED_EDGE('',*,*,#57186,.F.);
#81676=ORIENTED_EDGE('',*,*,#53843,.F.);
#81677=ORIENTED_EDGE('',*,*,#57185,.T.);
#81678=ORIENTED_EDGE('',*,*,#52208,.F.);
#81679=ORIENTED_EDGE('',*,*,#57187,.F.);
#81680=ORIENTED_EDGE('',*,*,#55293,.F.);
#81681=ORIENTED_EDGE('',*,*,#57186,.T.);
#81682=ORIENTED_EDGE('',*,*,#55312,.F.);
#81683=ORIENTED_EDGE('',*,*,#57188,.F.);
#81684=ORIENTED_EDGE('',*,*,#53861,.F.);
#81685=ORIENTED_EDGE('',*,*,#57187,.T.);
#81686=ORIENTED_EDGE('',*,*,#52207,.F.);
#81687=ORIENTED_EDGE('',*,*,#57189,.F.);
#81688=ORIENTED_EDGE('',*,*,#56390,.F.);
#81689=ORIENTED_EDGE('',*,*,#57188,.T.);
#81690=ORIENTED_EDGE('',*,*,#55311,.F.);
#81691=ORIENTED_EDGE('',*,*,#57190,.F.);
#81692=ORIENTED_EDGE('',*,*,#52456,.F.);
#81693=ORIENTED_EDGE('',*,*,#57189,.T.);
#81694=ORIENTED_EDGE('',*,*,#52206,.F.);
#81695=ORIENTED_EDGE('',*,*,#57191,.F.);
#81696=ORIENTED_EDGE('',*,*,#55299,.F.);
#81697=ORIENTED_EDGE('',*,*,#57190,.T.);
#81698=ORIENTED_EDGE('',*,*,#56389,.F.);
#81699=ORIENTED_EDGE('',*,*,#57192,.F.);
#81700=ORIENTED_EDGE('',*,*,#52457,.F.);
#81701=ORIENTED_EDGE('',*,*,#57191,.T.);
#81702=ORIENTED_EDGE('',*,*,#53892,.F.);
#81703=ORIENTED_EDGE('',*,*,#57193,.F.);
#81704=ORIENTED_EDGE('',*,*,#55300,.F.);
#81705=ORIENTED_EDGE('',*,*,#57192,.T.);
#81706=ORIENTED_EDGE('',*,*,#55295,.F.);
#81707=ORIENTED_EDGE('',*,*,#57194,.F.);
#81708=ORIENTED_EDGE('',*,*,#52458,.F.);
#81709=ORIENTED_EDGE('',*,*,#53887,.F.);
#81710=ORIENTED_EDGE('',*,*,#53883,.T.);
#81711=ORIENTED_EDGE('',*,*,#57195,.F.);
#81712=ORIENTED_EDGE('',*,*,#55301,.F.);
#81713=ORIENTED_EDGE('',*,*,#57193,.T.);
#81714=ORIENTED_EDGE('',*,*,#57194,.T.);
#81715=ORIENTED_EDGE('',*,*,#56391,.F.);
#81716=ORIENTED_EDGE('',*,*,#57196,.F.);
#81717=ORIENTED_EDGE('',*,*,#52459,.F.);
#81718=ORIENTED_EDGE('',*,*,#57195,.T.);
#81719=ORIENTED_EDGE('',*,*,#53882,.F.);
#81720=ORIENTED_EDGE('',*,*,#57197,.F.);
#81721=ORIENTED_EDGE('',*,*,#55302,.F.);
#81722=ORIENTED_EDGE('',*,*,#57196,.T.);
#81723=ORIENTED_EDGE('',*,*,#55297,.F.);
#81724=ORIENTED_EDGE('',*,*,#57198,.F.);
#81725=ORIENTED_EDGE('',*,*,#52460,.F.);
#81726=ORIENTED_EDGE('',*,*,#57197,.T.);
#81727=ORIENTED_EDGE('',*,*,#53894,.F.);
#81728=ORIENTED_EDGE('',*,*,#57199,.F.);
#81729=ORIENTED_EDGE('',*,*,#55303,.F.);
#81730=ORIENTED_EDGE('',*,*,#57198,.T.);
#81731=ORIENTED_EDGE('',*,*,#55296,.F.);
#81732=ORIENTED_EDGE('',*,*,#57200,.F.);
#81733=ORIENTED_EDGE('',*,*,#53890,.F.);
#81734=ORIENTED_EDGE('',*,*,#57199,.T.);
#81735=ORIENTED_EDGE('',*,*,#53878,.F.);
#81736=ORIENTED_EDGE('',*,*,#57201,.F.);
#81737=ORIENTED_EDGE('',*,*,#55304,.F.);
#81738=ORIENTED_EDGE('',*,*,#57200,.T.);
#81739=ORIENTED_EDGE('',*,*,#55307,.F.);
#81740=ORIENTED_EDGE('',*,*,#57202,.F.);
#81741=ORIENTED_EDGE('',*,*,#53869,.F.);
#81742=ORIENTED_EDGE('',*,*,#57201,.T.);
#81743=ORIENTED_EDGE('',*,*,#53896,.F.);
#81744=ORIENTED_EDGE('',*,*,#57203,.F.);
#81745=ORIENTED_EDGE('',*,*,#55305,.F.);
#81746=ORIENTED_EDGE('',*,*,#57202,.T.);
#81747=ORIENTED_EDGE('',*,*,#55306,.F.);
#81748=ORIENTED_EDGE('',*,*,#57203,.T.);
#81749=ORIENTED_EDGE('',*,*,#53874,.F.);
#81750=ORIENTED_EDGE('',*,*,#53870,.T.);
#81751=ORIENTED_EDGE('',*,*,#57204,.F.);
#81752=ORIENTED_EDGE('',*,*,#55346,.F.);
#81753=ORIENTED_EDGE('',*,*,#57205,.F.);
#81754=ORIENTED_EDGE('',*,*,#53826,.F.);
#81755=ORIENTED_EDGE('',*,*,#57205,.T.);
#81756=ORIENTED_EDGE('',*,*,#55345,.F.);
#81757=ORIENTED_EDGE('',*,*,#57206,.F.);
#81758=ORIENTED_EDGE('',*,*,#53835,.F.);
#81759=ORIENTED_EDGE('',*,*,#53825,.T.);
#81760=ORIENTED_EDGE('',*,*,#53829,.F.);
#81761=ORIENTED_EDGE('',*,*,#57207,.F.);
#81762=ORIENTED_EDGE('',*,*,#55347,.F.);
#81763=ORIENTED_EDGE('',*,*,#57204,.T.);
#81764=ORIENTED_EDGE('',*,*,#57206,.T.);
#81765=ORIENTED_EDGE('',*,*,#55344,.F.);
#81766=ORIENTED_EDGE('',*,*,#57208,.F.);
#81767=ORIENTED_EDGE('',*,*,#53820,.F.);
#81768=ORIENTED_EDGE('',*,*,#57207,.T.);
#81769=ORIENTED_EDGE('',*,*,#53833,.F.);
#81770=ORIENTED_EDGE('',*,*,#57209,.F.);
#81771=ORIENTED_EDGE('',*,*,#55336,.F.);
#81772=ORIENTED_EDGE('',*,*,#57208,.T.);
#81773=ORIENTED_EDGE('',*,*,#55343,.F.);
#81774=ORIENTED_EDGE('',*,*,#57210,.F.);
#81775=ORIENTED_EDGE('',*,*,#53837,.F.);
#81776=ORIENTED_EDGE('',*,*,#57209,.T.);
#81777=ORIENTED_EDGE('',*,*,#52216,.F.);
#81778=ORIENTED_EDGE('',*,*,#57211,.F.);
#81779=ORIENTED_EDGE('',*,*,#55337,.F.);
#81780=ORIENTED_EDGE('',*,*,#57210,.T.);
#81781=ORIENTED_EDGE('',*,*,#55342,.F.);
#81782=ORIENTED_EDGE('',*,*,#57212,.F.);
#81783=ORIENTED_EDGE('',*,*,#53812,.T.);
#81784=ORIENTED_EDGE('',*,*,#53816,.F.);
#81785=ORIENTED_EDGE('',*,*,#57211,.T.);
#81786=ORIENTED_EDGE('',*,*,#52215,.F.);
#81787=ORIENTED_EDGE('',*,*,#57213,.F.);
#81788=ORIENTED_EDGE('',*,*,#56392,.F.);
#81789=ORIENTED_EDGE('',*,*,#57212,.T.);
#81790=ORIENTED_EDGE('',*,*,#55341,.F.);
#81791=ORIENTED_EDGE('',*,*,#57214,.F.);
#81792=ORIENTED_EDGE('',*,*,#53813,.F.);
#81793=ORIENTED_EDGE('',*,*,#57213,.T.);
#81794=ORIENTED_EDGE('',*,*,#52214,.F.);
#81795=ORIENTED_EDGE('',*,*,#57215,.F.);
#81796=ORIENTED_EDGE('',*,*,#55321,.F.);
#81797=ORIENTED_EDGE('',*,*,#57214,.T.);
#81798=ORIENTED_EDGE('',*,*,#55340,.F.);
#81799=ORIENTED_EDGE('',*,*,#57216,.F.);
#81800=ORIENTED_EDGE('',*,*,#53831,.F.);
#81801=ORIENTED_EDGE('',*,*,#57215,.T.);
#81802=ORIENTED_EDGE('',*,*,#52213,.F.);
#81803=ORIENTED_EDGE('',*,*,#57217,.F.);
#81804=ORIENTED_EDGE('',*,*,#56394,.F.);
#81805=ORIENTED_EDGE('',*,*,#57216,.T.);
#81806=ORIENTED_EDGE('',*,*,#55339,.F.);
#81807=ORIENTED_EDGE('',*,*,#57218,.F.);
#81808=ORIENTED_EDGE('',*,*,#52450,.F.);
#81809=ORIENTED_EDGE('',*,*,#57217,.T.);
#81810=ORIENTED_EDGE('',*,*,#52212,.F.);
#81811=ORIENTED_EDGE('',*,*,#57219,.F.);
#81812=ORIENTED_EDGE('',*,*,#55327,.F.);
#81813=ORIENTED_EDGE('',*,*,#57218,.T.);
#81814=ORIENTED_EDGE('',*,*,#56393,.F.);
#81815=ORIENTED_EDGE('',*,*,#57220,.F.);
#81816=ORIENTED_EDGE('',*,*,#52451,.F.);
#81817=ORIENTED_EDGE('',*,*,#57219,.T.);
#81818=ORIENTED_EDGE('',*,*,#53862,.F.);
#81819=ORIENTED_EDGE('',*,*,#57221,.F.);
#81820=ORIENTED_EDGE('',*,*,#55328,.F.);
#81821=ORIENTED_EDGE('',*,*,#57220,.T.);
#81822=ORIENTED_EDGE('',*,*,#55323,.F.);
#81823=ORIENTED_EDGE('',*,*,#57222,.F.);
#81824=ORIENTED_EDGE('',*,*,#52452,.F.);
#81825=ORIENTED_EDGE('',*,*,#53857,.F.);
#81826=ORIENTED_EDGE('',*,*,#53853,.T.);
#81827=ORIENTED_EDGE('',*,*,#57223,.F.);
#81828=ORIENTED_EDGE('',*,*,#55329,.F.);
#81829=ORIENTED_EDGE('',*,*,#57221,.T.);
#81830=ORIENTED_EDGE('',*,*,#57222,.T.);
#81831=ORIENTED_EDGE('',*,*,#56395,.F.);
#81832=ORIENTED_EDGE('',*,*,#57224,.F.);
#81833=ORIENTED_EDGE('',*,*,#52453,.F.);
#81834=ORIENTED_EDGE('',*,*,#57223,.T.);
#81835=ORIENTED_EDGE('',*,*,#53852,.F.);
#81836=ORIENTED_EDGE('',*,*,#57225,.F.);
#81837=ORIENTED_EDGE('',*,*,#55330,.F.);
#81838=ORIENTED_EDGE('',*,*,#57224,.T.);
#81839=ORIENTED_EDGE('',*,*,#55325,.F.);
#81840=ORIENTED_EDGE('',*,*,#57226,.F.);
#81841=ORIENTED_EDGE('',*,*,#52454,.F.);
#81842=ORIENTED_EDGE('',*,*,#57225,.T.);
#81843=ORIENTED_EDGE('',*,*,#53864,.F.);
#81844=ORIENTED_EDGE('',*,*,#57227,.F.);
#81845=ORIENTED_EDGE('',*,*,#55331,.F.);
#81846=ORIENTED_EDGE('',*,*,#57226,.T.);
#81847=ORIENTED_EDGE('',*,*,#55324,.F.);
#81848=ORIENTED_EDGE('',*,*,#57228,.F.);
#81849=ORIENTED_EDGE('',*,*,#53860,.F.);
#81850=ORIENTED_EDGE('',*,*,#57227,.T.);
#81851=ORIENTED_EDGE('',*,*,#53848,.F.);
#81852=ORIENTED_EDGE('',*,*,#57229,.F.);
#81853=ORIENTED_EDGE('',*,*,#55332,.F.);
#81854=ORIENTED_EDGE('',*,*,#57228,.T.);
#81855=ORIENTED_EDGE('',*,*,#55335,.F.);
#81856=ORIENTED_EDGE('',*,*,#57230,.F.);
#81857=ORIENTED_EDGE('',*,*,#53839,.F.);
#81858=ORIENTED_EDGE('',*,*,#57229,.T.);
#81859=ORIENTED_EDGE('',*,*,#53866,.F.);
#81860=ORIENTED_EDGE('',*,*,#57231,.F.);
#81861=ORIENTED_EDGE('',*,*,#55333,.F.);
#81862=ORIENTED_EDGE('',*,*,#57230,.T.);
#81863=ORIENTED_EDGE('',*,*,#55334,.F.);
#81864=ORIENTED_EDGE('',*,*,#57231,.T.);
#81865=ORIENTED_EDGE('',*,*,#53844,.F.);
#81866=ORIENTED_EDGE('',*,*,#53840,.T.);
#81867=ORIENTED_EDGE('',*,*,#57232,.F.);
#81868=ORIENTED_EDGE('',*,*,#55374,.F.);
#81869=ORIENTED_EDGE('',*,*,#57233,.F.);
#81870=ORIENTED_EDGE('',*,*,#53796,.F.);
#81871=ORIENTED_EDGE('',*,*,#57233,.T.);
#81872=ORIENTED_EDGE('',*,*,#55373,.F.);
#81873=ORIENTED_EDGE('',*,*,#57234,.F.);
#81874=ORIENTED_EDGE('',*,*,#53805,.F.);
#81875=ORIENTED_EDGE('',*,*,#53795,.T.);
#81876=ORIENTED_EDGE('',*,*,#53799,.F.);
#81877=ORIENTED_EDGE('',*,*,#57235,.F.);
#81878=ORIENTED_EDGE('',*,*,#55375,.F.);
#81879=ORIENTED_EDGE('',*,*,#57232,.T.);
#81880=ORIENTED_EDGE('',*,*,#57234,.T.);
#81881=ORIENTED_EDGE('',*,*,#55372,.F.);
#81882=ORIENTED_EDGE('',*,*,#57236,.F.);
#81883=ORIENTED_EDGE('',*,*,#53790,.F.);
#81884=ORIENTED_EDGE('',*,*,#57235,.T.);
#81885=ORIENTED_EDGE('',*,*,#53803,.F.);
#81886=ORIENTED_EDGE('',*,*,#57237,.F.);
#81887=ORIENTED_EDGE('',*,*,#55364,.F.);
#81888=ORIENTED_EDGE('',*,*,#57236,.T.);
#81889=ORIENTED_EDGE('',*,*,#55371,.F.);
#81890=ORIENTED_EDGE('',*,*,#57238,.F.);
#81891=ORIENTED_EDGE('',*,*,#53807,.F.);
#81892=ORIENTED_EDGE('',*,*,#57237,.T.);
#81893=ORIENTED_EDGE('',*,*,#52222,.F.);
#81894=ORIENTED_EDGE('',*,*,#57239,.F.);
#81895=ORIENTED_EDGE('',*,*,#55365,.F.);
#81896=ORIENTED_EDGE('',*,*,#57238,.T.);
#81897=ORIENTED_EDGE('',*,*,#55370,.F.);
#81898=ORIENTED_EDGE('',*,*,#57240,.F.);
#81899=ORIENTED_EDGE('',*,*,#53782,.T.);
#81900=ORIENTED_EDGE('',*,*,#53786,.F.);
#81901=ORIENTED_EDGE('',*,*,#57239,.T.);
#81902=ORIENTED_EDGE('',*,*,#52221,.F.);
#81903=ORIENTED_EDGE('',*,*,#57241,.F.);
#81904=ORIENTED_EDGE('',*,*,#56396,.F.);
#81905=ORIENTED_EDGE('',*,*,#57240,.T.);
#81906=ORIENTED_EDGE('',*,*,#55369,.F.);
#81907=ORIENTED_EDGE('',*,*,#57242,.F.);
#81908=ORIENTED_EDGE('',*,*,#53783,.F.);
#81909=ORIENTED_EDGE('',*,*,#57241,.T.);
#81910=ORIENTED_EDGE('',*,*,#52220,.F.);
#81911=ORIENTED_EDGE('',*,*,#57243,.F.);
#81912=ORIENTED_EDGE('',*,*,#55349,.F.);
#81913=ORIENTED_EDGE('',*,*,#57242,.T.);
#81914=ORIENTED_EDGE('',*,*,#55368,.F.);
#81915=ORIENTED_EDGE('',*,*,#57244,.F.);
#81916=ORIENTED_EDGE('',*,*,#53801,.F.);
#81917=ORIENTED_EDGE('',*,*,#57243,.T.);
#81918=ORIENTED_EDGE('',*,*,#52219,.F.);
#81919=ORIENTED_EDGE('',*,*,#57245,.F.);
#81920=ORIENTED_EDGE('',*,*,#56398,.F.);
#81921=ORIENTED_EDGE('',*,*,#57244,.T.);
#81922=ORIENTED_EDGE('',*,*,#55367,.F.);
#81923=ORIENTED_EDGE('',*,*,#57246,.F.);
#81924=ORIENTED_EDGE('',*,*,#52444,.F.);
#81925=ORIENTED_EDGE('',*,*,#57245,.T.);
#81926=ORIENTED_EDGE('',*,*,#52218,.F.);
#81927=ORIENTED_EDGE('',*,*,#57247,.F.);
#81928=ORIENTED_EDGE('',*,*,#55355,.F.);
#81929=ORIENTED_EDGE('',*,*,#57246,.T.);
#81930=ORIENTED_EDGE('',*,*,#56397,.F.);
#81931=ORIENTED_EDGE('',*,*,#57248,.F.);
#81932=ORIENTED_EDGE('',*,*,#52445,.F.);
#81933=ORIENTED_EDGE('',*,*,#57247,.T.);
#81934=ORIENTED_EDGE('',*,*,#53832,.F.);
#81935=ORIENTED_EDGE('',*,*,#57249,.F.);
#81936=ORIENTED_EDGE('',*,*,#55356,.F.);
#81937=ORIENTED_EDGE('',*,*,#57248,.T.);
#81938=ORIENTED_EDGE('',*,*,#55351,.F.);
#81939=ORIENTED_EDGE('',*,*,#57250,.F.);
#81940=ORIENTED_EDGE('',*,*,#52446,.F.);
#81941=ORIENTED_EDGE('',*,*,#53827,.F.);
#81942=ORIENTED_EDGE('',*,*,#53823,.T.);
#81943=ORIENTED_EDGE('',*,*,#57251,.F.);
#81944=ORIENTED_EDGE('',*,*,#55357,.F.);
#81945=ORIENTED_EDGE('',*,*,#57249,.T.);
#81946=ORIENTED_EDGE('',*,*,#57250,.T.);
#81947=ORIENTED_EDGE('',*,*,#56399,.F.);
#81948=ORIENTED_EDGE('',*,*,#57252,.F.);
#81949=ORIENTED_EDGE('',*,*,#52447,.F.);
#81950=ORIENTED_EDGE('',*,*,#57251,.T.);
#81951=ORIENTED_EDGE('',*,*,#53822,.F.);
#81952=ORIENTED_EDGE('',*,*,#57253,.F.);
#81953=ORIENTED_EDGE('',*,*,#55358,.F.);
#81954=ORIENTED_EDGE('',*,*,#57252,.T.);
#81955=ORIENTED_EDGE('',*,*,#55353,.F.);
#81956=ORIENTED_EDGE('',*,*,#57254,.F.);
#81957=ORIENTED_EDGE('',*,*,#52448,.F.);
#81958=ORIENTED_EDGE('',*,*,#57253,.T.);
#81959=ORIENTED_EDGE('',*,*,#53834,.F.);
#81960=ORIENTED_EDGE('',*,*,#57255,.F.);
#81961=ORIENTED_EDGE('',*,*,#55359,.F.);
#81962=ORIENTED_EDGE('',*,*,#57254,.T.);
#81963=ORIENTED_EDGE('',*,*,#55352,.F.);
#81964=ORIENTED_EDGE('',*,*,#57256,.F.);
#81965=ORIENTED_EDGE('',*,*,#53830,.F.);
#81966=ORIENTED_EDGE('',*,*,#57255,.T.);
#81967=ORIENTED_EDGE('',*,*,#53818,.F.);
#81968=ORIENTED_EDGE('',*,*,#57257,.F.);
#81969=ORIENTED_EDGE('',*,*,#55360,.F.);
#81970=ORIENTED_EDGE('',*,*,#57256,.T.);
#81971=ORIENTED_EDGE('',*,*,#55363,.F.);
#81972=ORIENTED_EDGE('',*,*,#57258,.F.);
#81973=ORIENTED_EDGE('',*,*,#53809,.F.);
#81974=ORIENTED_EDGE('',*,*,#57257,.T.);
#81975=ORIENTED_EDGE('',*,*,#53836,.F.);
#81976=ORIENTED_EDGE('',*,*,#57259,.F.);
#81977=ORIENTED_EDGE('',*,*,#55361,.F.);
#81978=ORIENTED_EDGE('',*,*,#57258,.T.);
#81979=ORIENTED_EDGE('',*,*,#55362,.F.);
#81980=ORIENTED_EDGE('',*,*,#57259,.T.);
#81981=ORIENTED_EDGE('',*,*,#53814,.F.);
#81982=ORIENTED_EDGE('',*,*,#53810,.T.);
#81983=ORIENTED_EDGE('',*,*,#57260,.F.);
#81984=ORIENTED_EDGE('',*,*,#55402,.F.);
#81985=ORIENTED_EDGE('',*,*,#57261,.F.);
#81986=ORIENTED_EDGE('',*,*,#53766,.F.);
#81987=ORIENTED_EDGE('',*,*,#57261,.T.);
#81988=ORIENTED_EDGE('',*,*,#55401,.F.);
#81989=ORIENTED_EDGE('',*,*,#57262,.F.);
#81990=ORIENTED_EDGE('',*,*,#53775,.F.);
#81991=ORIENTED_EDGE('',*,*,#53765,.T.);
#81992=ORIENTED_EDGE('',*,*,#53769,.F.);
#81993=ORIENTED_EDGE('',*,*,#57263,.F.);
#81994=ORIENTED_EDGE('',*,*,#55403,.F.);
#81995=ORIENTED_EDGE('',*,*,#57260,.T.);
#81996=ORIENTED_EDGE('',*,*,#57262,.T.);
#81997=ORIENTED_EDGE('',*,*,#55400,.F.);
#81998=ORIENTED_EDGE('',*,*,#57264,.F.);
#81999=ORIENTED_EDGE('',*,*,#53760,.F.);
#82000=ORIENTED_EDGE('',*,*,#57263,.T.);
#82001=ORIENTED_EDGE('',*,*,#53773,.F.);
#82002=ORIENTED_EDGE('',*,*,#57265,.F.);
#82003=ORIENTED_EDGE('',*,*,#55392,.F.);
#82004=ORIENTED_EDGE('',*,*,#57264,.T.);
#82005=ORIENTED_EDGE('',*,*,#55399,.F.);
#82006=ORIENTED_EDGE('',*,*,#57266,.F.);
#82007=ORIENTED_EDGE('',*,*,#53777,.F.);
#82008=ORIENTED_EDGE('',*,*,#57265,.T.);
#82009=ORIENTED_EDGE('',*,*,#52228,.F.);
#82010=ORIENTED_EDGE('',*,*,#57267,.F.);
#82011=ORIENTED_EDGE('',*,*,#55393,.F.);
#82012=ORIENTED_EDGE('',*,*,#57266,.T.);
#82013=ORIENTED_EDGE('',*,*,#55398,.F.);
#82014=ORIENTED_EDGE('',*,*,#57268,.F.);
#82015=ORIENTED_EDGE('',*,*,#53752,.T.);
#82016=ORIENTED_EDGE('',*,*,#53756,.F.);
#82017=ORIENTED_EDGE('',*,*,#57267,.T.);
#82018=ORIENTED_EDGE('',*,*,#52227,.F.);
#82019=ORIENTED_EDGE('',*,*,#57269,.F.);
#82020=ORIENTED_EDGE('',*,*,#56400,.F.);
#82021=ORIENTED_EDGE('',*,*,#57268,.T.);
#82022=ORIENTED_EDGE('',*,*,#55397,.F.);
#82023=ORIENTED_EDGE('',*,*,#57270,.F.);
#82024=ORIENTED_EDGE('',*,*,#53753,.F.);
#82025=ORIENTED_EDGE('',*,*,#57269,.T.);
#82026=ORIENTED_EDGE('',*,*,#52226,.F.);
#82027=ORIENTED_EDGE('',*,*,#57271,.F.);
#82028=ORIENTED_EDGE('',*,*,#55377,.F.);
#82029=ORIENTED_EDGE('',*,*,#57270,.T.);
#82030=ORIENTED_EDGE('',*,*,#55396,.F.);
#82031=ORIENTED_EDGE('',*,*,#57272,.F.);
#82032=ORIENTED_EDGE('',*,*,#53771,.F.);
#82033=ORIENTED_EDGE('',*,*,#57271,.T.);
#82034=ORIENTED_EDGE('',*,*,#52225,.F.);
#82035=ORIENTED_EDGE('',*,*,#57273,.F.);
#82036=ORIENTED_EDGE('',*,*,#56402,.F.);
#82037=ORIENTED_EDGE('',*,*,#57272,.T.);
#82038=ORIENTED_EDGE('',*,*,#55395,.F.);
#82039=ORIENTED_EDGE('',*,*,#57274,.F.);
#82040=ORIENTED_EDGE('',*,*,#52438,.F.);
#82041=ORIENTED_EDGE('',*,*,#57273,.T.);
#82042=ORIENTED_EDGE('',*,*,#52224,.F.);
#82043=ORIENTED_EDGE('',*,*,#57275,.F.);
#82044=ORIENTED_EDGE('',*,*,#55383,.F.);
#82045=ORIENTED_EDGE('',*,*,#57274,.T.);
#82046=ORIENTED_EDGE('',*,*,#56401,.F.);
#82047=ORIENTED_EDGE('',*,*,#57276,.F.);
#82048=ORIENTED_EDGE('',*,*,#52439,.F.);
#82049=ORIENTED_EDGE('',*,*,#57275,.T.);
#82050=ORIENTED_EDGE('',*,*,#53802,.F.);
#82051=ORIENTED_EDGE('',*,*,#57277,.F.);
#82052=ORIENTED_EDGE('',*,*,#55384,.F.);
#82053=ORIENTED_EDGE('',*,*,#57276,.T.);
#82054=ORIENTED_EDGE('',*,*,#55379,.F.);
#82055=ORIENTED_EDGE('',*,*,#57278,.F.);
#82056=ORIENTED_EDGE('',*,*,#52440,.F.);
#82057=ORIENTED_EDGE('',*,*,#53797,.F.);
#82058=ORIENTED_EDGE('',*,*,#53793,.T.);
#82059=ORIENTED_EDGE('',*,*,#57279,.F.);
#82060=ORIENTED_EDGE('',*,*,#55385,.F.);
#82061=ORIENTED_EDGE('',*,*,#57277,.T.);
#82062=ORIENTED_EDGE('',*,*,#57278,.T.);
#82063=ORIENTED_EDGE('',*,*,#56403,.F.);
#82064=ORIENTED_EDGE('',*,*,#57280,.F.);
#82065=ORIENTED_EDGE('',*,*,#52441,.F.);
#82066=ORIENTED_EDGE('',*,*,#57279,.T.);
#82067=ORIENTED_EDGE('',*,*,#53792,.F.);
#82068=ORIENTED_EDGE('',*,*,#57281,.F.);
#82069=ORIENTED_EDGE('',*,*,#55386,.F.);
#82070=ORIENTED_EDGE('',*,*,#57280,.T.);
#82071=ORIENTED_EDGE('',*,*,#55381,.F.);
#82072=ORIENTED_EDGE('',*,*,#57282,.F.);
#82073=ORIENTED_EDGE('',*,*,#52442,.F.);
#82074=ORIENTED_EDGE('',*,*,#57281,.T.);
#82075=ORIENTED_EDGE('',*,*,#53804,.F.);
#82076=ORIENTED_EDGE('',*,*,#57283,.F.);
#82077=ORIENTED_EDGE('',*,*,#55387,.F.);
#82078=ORIENTED_EDGE('',*,*,#57282,.T.);
#82079=ORIENTED_EDGE('',*,*,#55380,.F.);
#82080=ORIENTED_EDGE('',*,*,#57284,.F.);
#82081=ORIENTED_EDGE('',*,*,#53800,.F.);
#82082=ORIENTED_EDGE('',*,*,#57283,.T.);
#82083=ORIENTED_EDGE('',*,*,#53788,.F.);
#82084=ORIENTED_EDGE('',*,*,#57285,.F.);
#82085=ORIENTED_EDGE('',*,*,#55388,.F.);
#82086=ORIENTED_EDGE('',*,*,#57284,.T.);
#82087=ORIENTED_EDGE('',*,*,#55391,.F.);
#82088=ORIENTED_EDGE('',*,*,#57286,.F.);
#82089=ORIENTED_EDGE('',*,*,#53779,.F.);
#82090=ORIENTED_EDGE('',*,*,#57285,.T.);
#82091=ORIENTED_EDGE('',*,*,#53806,.F.);
#82092=ORIENTED_EDGE('',*,*,#57287,.F.);
#82093=ORIENTED_EDGE('',*,*,#55389,.F.);
#82094=ORIENTED_EDGE('',*,*,#57286,.T.);
#82095=ORIENTED_EDGE('',*,*,#55390,.F.);
#82096=ORIENTED_EDGE('',*,*,#57287,.T.);
#82097=ORIENTED_EDGE('',*,*,#53784,.F.);
#82098=ORIENTED_EDGE('',*,*,#53780,.T.);
#82099=ORIENTED_EDGE('',*,*,#57288,.F.);
#82100=ORIENTED_EDGE('',*,*,#55430,.F.);
#82101=ORIENTED_EDGE('',*,*,#57289,.F.);
#82102=ORIENTED_EDGE('',*,*,#53736,.F.);
#82103=ORIENTED_EDGE('',*,*,#57289,.T.);
#82104=ORIENTED_EDGE('',*,*,#55429,.F.);
#82105=ORIENTED_EDGE('',*,*,#57290,.F.);
#82106=ORIENTED_EDGE('',*,*,#53745,.F.);
#82107=ORIENTED_EDGE('',*,*,#53735,.T.);
#82108=ORIENTED_EDGE('',*,*,#53739,.F.);
#82109=ORIENTED_EDGE('',*,*,#57291,.F.);
#82110=ORIENTED_EDGE('',*,*,#55431,.F.);
#82111=ORIENTED_EDGE('',*,*,#57288,.T.);
#82112=ORIENTED_EDGE('',*,*,#57290,.T.);
#82113=ORIENTED_EDGE('',*,*,#55428,.F.);
#82114=ORIENTED_EDGE('',*,*,#57292,.F.);
#82115=ORIENTED_EDGE('',*,*,#53730,.F.);
#82116=ORIENTED_EDGE('',*,*,#57291,.T.);
#82117=ORIENTED_EDGE('',*,*,#53743,.F.);
#82118=ORIENTED_EDGE('',*,*,#57293,.F.);
#82119=ORIENTED_EDGE('',*,*,#55420,.F.);
#82120=ORIENTED_EDGE('',*,*,#57292,.T.);
#82121=ORIENTED_EDGE('',*,*,#55427,.F.);
#82122=ORIENTED_EDGE('',*,*,#57294,.F.);
#82123=ORIENTED_EDGE('',*,*,#53747,.F.);
#82124=ORIENTED_EDGE('',*,*,#57293,.T.);
#82125=ORIENTED_EDGE('',*,*,#52234,.F.);
#82126=ORIENTED_EDGE('',*,*,#57295,.F.);
#82127=ORIENTED_EDGE('',*,*,#55421,.F.);
#82128=ORIENTED_EDGE('',*,*,#57294,.T.);
#82129=ORIENTED_EDGE('',*,*,#55426,.F.);
#82130=ORIENTED_EDGE('',*,*,#57296,.F.);
#82131=ORIENTED_EDGE('',*,*,#53722,.T.);
#82132=ORIENTED_EDGE('',*,*,#53726,.F.);
#82133=ORIENTED_EDGE('',*,*,#57295,.T.);
#82134=ORIENTED_EDGE('',*,*,#52233,.F.);
#82135=ORIENTED_EDGE('',*,*,#57297,.F.);
#82136=ORIENTED_EDGE('',*,*,#56404,.F.);
#82137=ORIENTED_EDGE('',*,*,#57296,.T.);
#82138=ORIENTED_EDGE('',*,*,#55425,.F.);
#82139=ORIENTED_EDGE('',*,*,#57298,.F.);
#82140=ORIENTED_EDGE('',*,*,#53723,.F.);
#82141=ORIENTED_EDGE('',*,*,#57297,.T.);
#82142=ORIENTED_EDGE('',*,*,#52232,.F.);
#82143=ORIENTED_EDGE('',*,*,#57299,.F.);
#82144=ORIENTED_EDGE('',*,*,#55405,.F.);
#82145=ORIENTED_EDGE('',*,*,#57298,.T.);
#82146=ORIENTED_EDGE('',*,*,#55424,.F.);
#82147=ORIENTED_EDGE('',*,*,#57300,.F.);
#82148=ORIENTED_EDGE('',*,*,#53741,.F.);
#82149=ORIENTED_EDGE('',*,*,#57299,.T.);
#82150=ORIENTED_EDGE('',*,*,#52231,.F.);
#82151=ORIENTED_EDGE('',*,*,#57301,.F.);
#82152=ORIENTED_EDGE('',*,*,#56406,.F.);
#82153=ORIENTED_EDGE('',*,*,#57300,.T.);
#82154=ORIENTED_EDGE('',*,*,#55423,.F.);
#82155=ORIENTED_EDGE('',*,*,#57302,.F.);
#82156=ORIENTED_EDGE('',*,*,#52432,.F.);
#82157=ORIENTED_EDGE('',*,*,#57301,.T.);
#82158=ORIENTED_EDGE('',*,*,#52230,.F.);
#82159=ORIENTED_EDGE('',*,*,#57303,.F.);
#82160=ORIENTED_EDGE('',*,*,#55411,.F.);
#82161=ORIENTED_EDGE('',*,*,#57302,.T.);
#82162=ORIENTED_EDGE('',*,*,#56405,.F.);
#82163=ORIENTED_EDGE('',*,*,#57304,.F.);
#82164=ORIENTED_EDGE('',*,*,#52433,.F.);
#82165=ORIENTED_EDGE('',*,*,#57303,.T.);
#82166=ORIENTED_EDGE('',*,*,#53772,.F.);
#82167=ORIENTED_EDGE('',*,*,#57305,.F.);
#82168=ORIENTED_EDGE('',*,*,#55412,.F.);
#82169=ORIENTED_EDGE('',*,*,#57304,.T.);
#82170=ORIENTED_EDGE('',*,*,#55407,.F.);
#82171=ORIENTED_EDGE('',*,*,#57306,.F.);
#82172=ORIENTED_EDGE('',*,*,#52434,.F.);
#82173=ORIENTED_EDGE('',*,*,#53767,.F.);
#82174=ORIENTED_EDGE('',*,*,#53763,.T.);
#82175=ORIENTED_EDGE('',*,*,#57307,.F.);
#82176=ORIENTED_EDGE('',*,*,#55413,.F.);
#82177=ORIENTED_EDGE('',*,*,#57305,.T.);
#82178=ORIENTED_EDGE('',*,*,#57306,.T.);
#82179=ORIENTED_EDGE('',*,*,#56407,.F.);
#82180=ORIENTED_EDGE('',*,*,#57308,.F.);
#82181=ORIENTED_EDGE('',*,*,#52435,.F.);
#82182=ORIENTED_EDGE('',*,*,#57307,.T.);
#82183=ORIENTED_EDGE('',*,*,#53762,.F.);
#82184=ORIENTED_EDGE('',*,*,#57309,.F.);
#82185=ORIENTED_EDGE('',*,*,#55414,.F.);
#82186=ORIENTED_EDGE('',*,*,#57308,.T.);
#82187=ORIENTED_EDGE('',*,*,#55409,.F.);
#82188=ORIENTED_EDGE('',*,*,#57310,.F.);
#82189=ORIENTED_EDGE('',*,*,#52436,.F.);
#82190=ORIENTED_EDGE('',*,*,#57309,.T.);
#82191=ORIENTED_EDGE('',*,*,#53774,.F.);
#82192=ORIENTED_EDGE('',*,*,#57311,.F.);
#82193=ORIENTED_EDGE('',*,*,#55415,.F.);
#82194=ORIENTED_EDGE('',*,*,#57310,.T.);
#82195=ORIENTED_EDGE('',*,*,#55408,.F.);
#82196=ORIENTED_EDGE('',*,*,#57312,.F.);
#82197=ORIENTED_EDGE('',*,*,#53770,.F.);
#82198=ORIENTED_EDGE('',*,*,#57311,.T.);
#82199=ORIENTED_EDGE('',*,*,#53758,.F.);
#82200=ORIENTED_EDGE('',*,*,#57313,.F.);
#82201=ORIENTED_EDGE('',*,*,#55416,.F.);
#82202=ORIENTED_EDGE('',*,*,#57312,.T.);
#82203=ORIENTED_EDGE('',*,*,#55419,.F.);
#82204=ORIENTED_EDGE('',*,*,#57314,.F.);
#82205=ORIENTED_EDGE('',*,*,#53749,.F.);
#82206=ORIENTED_EDGE('',*,*,#57313,.T.);
#82207=ORIENTED_EDGE('',*,*,#53776,.F.);
#82208=ORIENTED_EDGE('',*,*,#57315,.F.);
#82209=ORIENTED_EDGE('',*,*,#55417,.F.);
#82210=ORIENTED_EDGE('',*,*,#57314,.T.);
#82211=ORIENTED_EDGE('',*,*,#55418,.F.);
#82212=ORIENTED_EDGE('',*,*,#57315,.T.);
#82213=ORIENTED_EDGE('',*,*,#53754,.F.);
#82214=ORIENTED_EDGE('',*,*,#53750,.T.);
#82215=ORIENTED_EDGE('',*,*,#57316,.F.);
#82216=ORIENTED_EDGE('',*,*,#55458,.F.);
#82217=ORIENTED_EDGE('',*,*,#57317,.F.);
#82218=ORIENTED_EDGE('',*,*,#53706,.F.);
#82219=ORIENTED_EDGE('',*,*,#57317,.T.);
#82220=ORIENTED_EDGE('',*,*,#55457,.F.);
#82221=ORIENTED_EDGE('',*,*,#57318,.F.);
#82222=ORIENTED_EDGE('',*,*,#53715,.F.);
#82223=ORIENTED_EDGE('',*,*,#53705,.T.);
#82224=ORIENTED_EDGE('',*,*,#53709,.F.);
#82225=ORIENTED_EDGE('',*,*,#57319,.F.);
#82226=ORIENTED_EDGE('',*,*,#55459,.F.);
#82227=ORIENTED_EDGE('',*,*,#57316,.T.);
#82228=ORIENTED_EDGE('',*,*,#57318,.T.);
#82229=ORIENTED_EDGE('',*,*,#55456,.F.);
#82230=ORIENTED_EDGE('',*,*,#57320,.F.);
#82231=ORIENTED_EDGE('',*,*,#53700,.F.);
#82232=ORIENTED_EDGE('',*,*,#57319,.T.);
#82233=ORIENTED_EDGE('',*,*,#53713,.F.);
#82234=ORIENTED_EDGE('',*,*,#57321,.F.);
#82235=ORIENTED_EDGE('',*,*,#55448,.F.);
#82236=ORIENTED_EDGE('',*,*,#57320,.T.);
#82237=ORIENTED_EDGE('',*,*,#55455,.F.);
#82238=ORIENTED_EDGE('',*,*,#57322,.F.);
#82239=ORIENTED_EDGE('',*,*,#53717,.F.);
#82240=ORIENTED_EDGE('',*,*,#57321,.T.);
#82241=ORIENTED_EDGE('',*,*,#52240,.F.);
#82242=ORIENTED_EDGE('',*,*,#57323,.F.);
#82243=ORIENTED_EDGE('',*,*,#55449,.F.);
#82244=ORIENTED_EDGE('',*,*,#57322,.T.);
#82245=ORIENTED_EDGE('',*,*,#55454,.F.);
#82246=ORIENTED_EDGE('',*,*,#57324,.F.);
#82247=ORIENTED_EDGE('',*,*,#53692,.T.);
#82248=ORIENTED_EDGE('',*,*,#53696,.F.);
#82249=ORIENTED_EDGE('',*,*,#57323,.T.);
#82250=ORIENTED_EDGE('',*,*,#52239,.F.);
#82251=ORIENTED_EDGE('',*,*,#57325,.F.);
#82252=ORIENTED_EDGE('',*,*,#56408,.F.);
#82253=ORIENTED_EDGE('',*,*,#57324,.T.);
#82254=ORIENTED_EDGE('',*,*,#55453,.F.);
#82255=ORIENTED_EDGE('',*,*,#57326,.F.);
#82256=ORIENTED_EDGE('',*,*,#53693,.F.);
#82257=ORIENTED_EDGE('',*,*,#57325,.T.);
#82258=ORIENTED_EDGE('',*,*,#52238,.F.);
#82259=ORIENTED_EDGE('',*,*,#57327,.F.);
#82260=ORIENTED_EDGE('',*,*,#55433,.F.);
#82261=ORIENTED_EDGE('',*,*,#57326,.T.);
#82262=ORIENTED_EDGE('',*,*,#55452,.F.);
#82263=ORIENTED_EDGE('',*,*,#57328,.F.);
#82264=ORIENTED_EDGE('',*,*,#53711,.F.);
#82265=ORIENTED_EDGE('',*,*,#57327,.T.);
#82266=ORIENTED_EDGE('',*,*,#52237,.F.);
#82267=ORIENTED_EDGE('',*,*,#57329,.F.);
#82268=ORIENTED_EDGE('',*,*,#56410,.F.);
#82269=ORIENTED_EDGE('',*,*,#57328,.T.);
#82270=ORIENTED_EDGE('',*,*,#55451,.F.);
#82271=ORIENTED_EDGE('',*,*,#57330,.F.);
#82272=ORIENTED_EDGE('',*,*,#52426,.F.);
#82273=ORIENTED_EDGE('',*,*,#57329,.T.);
#82274=ORIENTED_EDGE('',*,*,#52236,.F.);
#82275=ORIENTED_EDGE('',*,*,#57331,.F.);
#82276=ORIENTED_EDGE('',*,*,#55439,.F.);
#82277=ORIENTED_EDGE('',*,*,#57330,.T.);
#82278=ORIENTED_EDGE('',*,*,#56409,.F.);
#82279=ORIENTED_EDGE('',*,*,#57332,.F.);
#82280=ORIENTED_EDGE('',*,*,#52427,.F.);
#82281=ORIENTED_EDGE('',*,*,#57331,.T.);
#82282=ORIENTED_EDGE('',*,*,#53742,.F.);
#82283=ORIENTED_EDGE('',*,*,#57333,.F.);
#82284=ORIENTED_EDGE('',*,*,#55440,.F.);
#82285=ORIENTED_EDGE('',*,*,#57332,.T.);
#82286=ORIENTED_EDGE('',*,*,#55435,.F.);
#82287=ORIENTED_EDGE('',*,*,#57334,.F.);
#82288=ORIENTED_EDGE('',*,*,#52428,.F.);
#82289=ORIENTED_EDGE('',*,*,#53737,.F.);
#82290=ORIENTED_EDGE('',*,*,#53733,.T.);
#82291=ORIENTED_EDGE('',*,*,#57335,.F.);
#82292=ORIENTED_EDGE('',*,*,#55441,.F.);
#82293=ORIENTED_EDGE('',*,*,#57333,.T.);
#82294=ORIENTED_EDGE('',*,*,#57334,.T.);
#82295=ORIENTED_EDGE('',*,*,#56411,.F.);
#82296=ORIENTED_EDGE('',*,*,#57336,.F.);
#82297=ORIENTED_EDGE('',*,*,#52429,.F.);
#82298=ORIENTED_EDGE('',*,*,#57335,.T.);
#82299=ORIENTED_EDGE('',*,*,#53732,.F.);
#82300=ORIENTED_EDGE('',*,*,#57337,.F.);
#82301=ORIENTED_EDGE('',*,*,#55442,.F.);
#82302=ORIENTED_EDGE('',*,*,#57336,.T.);
#82303=ORIENTED_EDGE('',*,*,#55437,.F.);
#82304=ORIENTED_EDGE('',*,*,#57338,.F.);
#82305=ORIENTED_EDGE('',*,*,#52430,.F.);
#82306=ORIENTED_EDGE('',*,*,#57337,.T.);
#82307=ORIENTED_EDGE('',*,*,#53744,.F.);
#82308=ORIENTED_EDGE('',*,*,#57339,.F.);
#82309=ORIENTED_EDGE('',*,*,#55443,.F.);
#82310=ORIENTED_EDGE('',*,*,#57338,.T.);
#82311=ORIENTED_EDGE('',*,*,#55436,.F.);
#82312=ORIENTED_EDGE('',*,*,#57340,.F.);
#82313=ORIENTED_EDGE('',*,*,#53740,.F.);
#82314=ORIENTED_EDGE('',*,*,#57339,.T.);
#82315=ORIENTED_EDGE('',*,*,#53728,.F.);
#82316=ORIENTED_EDGE('',*,*,#57341,.F.);
#82317=ORIENTED_EDGE('',*,*,#55444,.F.);
#82318=ORIENTED_EDGE('',*,*,#57340,.T.);
#82319=ORIENTED_EDGE('',*,*,#55447,.F.);
#82320=ORIENTED_EDGE('',*,*,#57342,.F.);
#82321=ORIENTED_EDGE('',*,*,#53719,.F.);
#82322=ORIENTED_EDGE('',*,*,#57341,.T.);
#82323=ORIENTED_EDGE('',*,*,#53746,.F.);
#82324=ORIENTED_EDGE('',*,*,#57343,.F.);
#82325=ORIENTED_EDGE('',*,*,#55445,.F.);
#82326=ORIENTED_EDGE('',*,*,#57342,.T.);
#82327=ORIENTED_EDGE('',*,*,#55446,.F.);
#82328=ORIENTED_EDGE('',*,*,#57343,.T.);
#82329=ORIENTED_EDGE('',*,*,#53724,.F.);
#82330=ORIENTED_EDGE('',*,*,#53720,.T.);
#82331=ORIENTED_EDGE('',*,*,#57344,.F.);
#82332=ORIENTED_EDGE('',*,*,#55484,.F.);
#82333=ORIENTED_EDGE('',*,*,#57345,.F.);
#82334=ORIENTED_EDGE('',*,*,#53676,.F.);
#82335=ORIENTED_EDGE('',*,*,#57345,.T.);
#82336=ORIENTED_EDGE('',*,*,#55483,.F.);
#82337=ORIENTED_EDGE('',*,*,#57346,.F.);
#82338=ORIENTED_EDGE('',*,*,#53685,.F.);
#82339=ORIENTED_EDGE('',*,*,#53675,.T.);
#82340=ORIENTED_EDGE('',*,*,#53679,.F.);
#82341=ORIENTED_EDGE('',*,*,#57347,.F.);
#82342=ORIENTED_EDGE('',*,*,#55485,.F.);
#82343=ORIENTED_EDGE('',*,*,#57344,.T.);
#82344=ORIENTED_EDGE('',*,*,#57346,.T.);
#82345=ORIENTED_EDGE('',*,*,#55482,.F.);
#82346=ORIENTED_EDGE('',*,*,#57348,.F.);
#82347=ORIENTED_EDGE('',*,*,#53670,.F.);
#82348=ORIENTED_EDGE('',*,*,#57347,.T.);
#82349=ORIENTED_EDGE('',*,*,#53683,.F.);
#82350=ORIENTED_EDGE('',*,*,#57349,.F.);
#82351=ORIENTED_EDGE('',*,*,#55474,.F.);
#82352=ORIENTED_EDGE('',*,*,#57348,.T.);
#82353=ORIENTED_EDGE('',*,*,#55481,.F.);
#82354=ORIENTED_EDGE('',*,*,#57350,.F.);
#82355=ORIENTED_EDGE('',*,*,#53687,.F.);
#82356=ORIENTED_EDGE('',*,*,#57349,.T.);
#82357=ORIENTED_EDGE('',*,*,#52246,.F.);
#82358=ORIENTED_EDGE('',*,*,#57351,.F.);
#82359=ORIENTED_EDGE('',*,*,#55475,.F.);
#82360=ORIENTED_EDGE('',*,*,#57350,.T.);
#82361=ORIENTED_EDGE('',*,*,#55480,.F.);
#82362=ORIENTED_EDGE('',*,*,#57352,.F.);
#82363=ORIENTED_EDGE('',*,*,#53662,.T.);
#82364=ORIENTED_EDGE('',*,*,#53666,.F.);
#82365=ORIENTED_EDGE('',*,*,#57351,.T.);
#82366=ORIENTED_EDGE('',*,*,#52245,.F.);
#82367=ORIENTED_EDGE('',*,*,#52044,.F.);
#82368=ORIENTED_EDGE('',*,*,#56412,.F.);
#82369=ORIENTED_EDGE('',*,*,#57352,.T.);
#82370=ORIENTED_EDGE('',*,*,#55479,.F.);
#82371=ORIENTED_EDGE('',*,*,#57353,.F.);
#82372=ORIENTED_EDGE('',*,*,#53663,.F.);
#82373=ORIENTED_EDGE('',*,*,#57353,.T.);
#82374=ORIENTED_EDGE('',*,*,#55478,.F.);
#82375=ORIENTED_EDGE('',*,*,#57354,.F.);
#82376=ORIENTED_EDGE('',*,*,#53681,.F.);
#82377=ORIENTED_EDGE('',*,*,#52042,.T.);
#82378=ORIENTED_EDGE('',*,*,#52243,.F.);
#82379=ORIENTED_EDGE('',*,*,#57355,.F.);
#82380=ORIENTED_EDGE('',*,*,#56414,.F.);
#82381=ORIENTED_EDGE('',*,*,#57354,.T.);
#82382=ORIENTED_EDGE('',*,*,#55477,.F.);
#82383=ORIENTED_EDGE('',*,*,#57356,.F.);
#82384=ORIENTED_EDGE('',*,*,#52781,.F.);
#82385=ORIENTED_EDGE('',*,*,#57355,.T.);
#82386=ORIENTED_EDGE('',*,*,#52242,.F.);
#82387=ORIENTED_EDGE('',*,*,#57357,.F.);
#82388=ORIENTED_EDGE('',*,*,#55465,.F.);
#82389=ORIENTED_EDGE('',*,*,#57356,.T.);
#82390=ORIENTED_EDGE('',*,*,#56413,.F.);
#82391=ORIENTED_EDGE('',*,*,#52040,.F.);
#82392=ORIENTED_EDGE('',*,*,#52782,.F.);
#82393=ORIENTED_EDGE('',*,*,#57357,.T.);
#82394=ORIENTED_EDGE('',*,*,#53712,.F.);
#82395=ORIENTED_EDGE('',*,*,#57358,.F.);
#82396=ORIENTED_EDGE('',*,*,#55466,.F.);
#82397=ORIENTED_EDGE('',*,*,#53707,.F.);
#82398=ORIENTED_EDGE('',*,*,#53703,.T.);
#82399=ORIENTED_EDGE('',*,*,#57359,.F.);
#82400=ORIENTED_EDGE('',*,*,#55467,.F.);
#82401=ORIENTED_EDGE('',*,*,#57358,.T.);
#82402=ORIENTED_EDGE('',*,*,#52038,.T.);
#82403=ORIENTED_EDGE('',*,*,#56415,.F.);
#82404=ORIENTED_EDGE('',*,*,#57360,.F.);
#82405=ORIENTED_EDGE('',*,*,#52423,.F.);
#82406=ORIENTED_EDGE('',*,*,#57359,.T.);
#82407=ORIENTED_EDGE('',*,*,#53702,.F.);
#82408=ORIENTED_EDGE('',*,*,#57361,.F.);
#82409=ORIENTED_EDGE('',*,*,#55468,.F.);
#82410=ORIENTED_EDGE('',*,*,#57360,.T.);
#82411=ORIENTED_EDGE('',*,*,#55463,.F.);
#82412=ORIENTED_EDGE('',*,*,#57362,.F.);
#82413=ORIENTED_EDGE('',*,*,#52424,.F.);
#82414=ORIENTED_EDGE('',*,*,#57361,.T.);
#82415=ORIENTED_EDGE('',*,*,#53714,.F.);
#82416=ORIENTED_EDGE('',*,*,#57363,.F.);
#82417=ORIENTED_EDGE('',*,*,#55469,.F.);
#82418=ORIENTED_EDGE('',*,*,#57362,.T.);
#82419=ORIENTED_EDGE('',*,*,#55462,.F.);
#82420=ORIENTED_EDGE('',*,*,#57364,.F.);
#82421=ORIENTED_EDGE('',*,*,#53710,.F.);
#82422=ORIENTED_EDGE('',*,*,#57363,.T.);
#82423=ORIENTED_EDGE('',*,*,#53698,.F.);
#82424=ORIENTED_EDGE('',*,*,#57365,.F.);
#82425=ORIENTED_EDGE('',*,*,#55470,.F.);
#82426=ORIENTED_EDGE('',*,*,#57364,.T.);
#82427=ORIENTED_EDGE('',*,*,#55473,.F.);
#82428=ORIENTED_EDGE('',*,*,#57366,.F.);
#82429=ORIENTED_EDGE('',*,*,#53689,.F.);
#82430=ORIENTED_EDGE('',*,*,#57365,.T.);
#82431=ORIENTED_EDGE('',*,*,#53716,.F.);
#82432=ORIENTED_EDGE('',*,*,#57367,.F.);
#82433=ORIENTED_EDGE('',*,*,#55471,.F.);
#82434=ORIENTED_EDGE('',*,*,#57366,.T.);
#82435=ORIENTED_EDGE('',*,*,#55472,.F.);
#82436=ORIENTED_EDGE('',*,*,#57367,.T.);
#82437=ORIENTED_EDGE('',*,*,#53694,.F.);
#82438=ORIENTED_EDGE('',*,*,#53690,.T.);
#82439=ORIENTED_EDGE('',*,*,#57368,.F.);
#82440=ORIENTED_EDGE('',*,*,#55512,.F.);
#82441=ORIENTED_EDGE('',*,*,#57369,.F.);
#82442=ORIENTED_EDGE('',*,*,#53646,.F.);
#82443=ORIENTED_EDGE('',*,*,#57369,.T.);
#82444=ORIENTED_EDGE('',*,*,#55511,.F.);
#82445=ORIENTED_EDGE('',*,*,#57370,.F.);
#82446=ORIENTED_EDGE('',*,*,#53655,.F.);
#82447=ORIENTED_EDGE('',*,*,#53645,.T.);
#82448=ORIENTED_EDGE('',*,*,#53649,.F.);
#82449=ORIENTED_EDGE('',*,*,#57371,.F.);
#82450=ORIENTED_EDGE('',*,*,#55513,.F.);
#82451=ORIENTED_EDGE('',*,*,#57368,.T.);
#82452=ORIENTED_EDGE('',*,*,#57370,.T.);
#82453=ORIENTED_EDGE('',*,*,#55510,.F.);
#82454=ORIENTED_EDGE('',*,*,#57372,.F.);
#82455=ORIENTED_EDGE('',*,*,#53640,.F.);
#82456=ORIENTED_EDGE('',*,*,#57371,.T.);
#82457=ORIENTED_EDGE('',*,*,#53653,.F.);
#82458=ORIENTED_EDGE('',*,*,#57373,.F.);
#82459=ORIENTED_EDGE('',*,*,#55502,.F.);
#82460=ORIENTED_EDGE('',*,*,#57372,.T.);
#82461=ORIENTED_EDGE('',*,*,#55509,.F.);
#82462=ORIENTED_EDGE('',*,*,#57374,.F.);
#82463=ORIENTED_EDGE('',*,*,#53657,.F.);
#82464=ORIENTED_EDGE('',*,*,#57373,.T.);
#82465=ORIENTED_EDGE('',*,*,#52252,.F.);
#82466=ORIENTED_EDGE('',*,*,#57375,.F.);
#82467=ORIENTED_EDGE('',*,*,#55503,.F.);
#82468=ORIENTED_EDGE('',*,*,#57374,.T.);
#82469=ORIENTED_EDGE('',*,*,#55508,.F.);
#82470=ORIENTED_EDGE('',*,*,#57376,.F.);
#82471=ORIENTED_EDGE('',*,*,#53632,.T.);
#82472=ORIENTED_EDGE('',*,*,#53636,.F.);
#82473=ORIENTED_EDGE('',*,*,#57375,.T.);
#82474=ORIENTED_EDGE('',*,*,#52251,.F.);
#82475=ORIENTED_EDGE('',*,*,#57377,.F.);
#82476=ORIENTED_EDGE('',*,*,#56416,.F.);
#82477=ORIENTED_EDGE('',*,*,#57376,.T.);
#82478=ORIENTED_EDGE('',*,*,#55507,.F.);
#82479=ORIENTED_EDGE('',*,*,#57378,.F.);
#82480=ORIENTED_EDGE('',*,*,#53633,.F.);
#82481=ORIENTED_EDGE('',*,*,#57377,.T.);
#82482=ORIENTED_EDGE('',*,*,#52250,.F.);
#82483=ORIENTED_EDGE('',*,*,#57379,.F.);
#82484=ORIENTED_EDGE('',*,*,#55487,.F.);
#82485=ORIENTED_EDGE('',*,*,#57378,.T.);
#82486=ORIENTED_EDGE('',*,*,#55506,.F.);
#82487=ORIENTED_EDGE('',*,*,#57380,.F.);
#82488=ORIENTED_EDGE('',*,*,#53651,.F.);
#82489=ORIENTED_EDGE('',*,*,#57379,.T.);
#82490=ORIENTED_EDGE('',*,*,#52249,.F.);
#82491=ORIENTED_EDGE('',*,*,#57381,.F.);
#82492=ORIENTED_EDGE('',*,*,#56418,.F.);
#82493=ORIENTED_EDGE('',*,*,#57380,.T.);
#82494=ORIENTED_EDGE('',*,*,#55505,.F.);
#82495=ORIENTED_EDGE('',*,*,#57382,.F.);
#82496=ORIENTED_EDGE('',*,*,#52775,.F.);
#82497=ORIENTED_EDGE('',*,*,#57381,.T.);
#82498=ORIENTED_EDGE('',*,*,#52248,.F.);
#82499=ORIENTED_EDGE('',*,*,#57383,.F.);
#82500=ORIENTED_EDGE('',*,*,#55493,.F.);
#82501=ORIENTED_EDGE('',*,*,#57382,.T.);
#82502=ORIENTED_EDGE('',*,*,#56417,.F.);
#82503=ORIENTED_EDGE('',*,*,#57384,.F.);
#82504=ORIENTED_EDGE('',*,*,#52776,.F.);
#82505=ORIENTED_EDGE('',*,*,#57383,.T.);
#82506=ORIENTED_EDGE('',*,*,#53682,.F.);
#82507=ORIENTED_EDGE('',*,*,#57385,.F.);
#82508=ORIENTED_EDGE('',*,*,#55494,.F.);
#82509=ORIENTED_EDGE('',*,*,#57384,.T.);
#82510=ORIENTED_EDGE('',*,*,#55489,.F.);
#82511=ORIENTED_EDGE('',*,*,#57386,.F.);
#82512=ORIENTED_EDGE('',*,*,#52777,.F.);
#82513=ORIENTED_EDGE('',*,*,#53677,.F.);
#82514=ORIENTED_EDGE('',*,*,#53673,.T.);
#82515=ORIENTED_EDGE('',*,*,#57387,.F.);
#82516=ORIENTED_EDGE('',*,*,#55495,.F.);
#82517=ORIENTED_EDGE('',*,*,#57385,.T.);
#82518=ORIENTED_EDGE('',*,*,#57386,.T.);
#82519=ORIENTED_EDGE('',*,*,#56419,.F.);
#82520=ORIENTED_EDGE('',*,*,#57388,.F.);
#82521=ORIENTED_EDGE('',*,*,#52778,.F.);
#82522=ORIENTED_EDGE('',*,*,#57387,.T.);
#82523=ORIENTED_EDGE('',*,*,#53672,.F.);
#82524=ORIENTED_EDGE('',*,*,#57389,.F.);
#82525=ORIENTED_EDGE('',*,*,#55496,.F.);
#82526=ORIENTED_EDGE('',*,*,#57388,.T.);
#82527=ORIENTED_EDGE('',*,*,#55491,.F.);
#82528=ORIENTED_EDGE('',*,*,#57390,.F.);
#82529=ORIENTED_EDGE('',*,*,#52779,.F.);
#82530=ORIENTED_EDGE('',*,*,#57389,.T.);
#82531=ORIENTED_EDGE('',*,*,#53684,.F.);
#82532=ORIENTED_EDGE('',*,*,#57391,.F.);
#82533=ORIENTED_EDGE('',*,*,#55497,.F.);
#82534=ORIENTED_EDGE('',*,*,#57390,.T.);
#82535=ORIENTED_EDGE('',*,*,#55490,.F.);
#82536=ORIENTED_EDGE('',*,*,#57392,.F.);
#82537=ORIENTED_EDGE('',*,*,#53680,.F.);
#82538=ORIENTED_EDGE('',*,*,#57391,.T.);
#82539=ORIENTED_EDGE('',*,*,#53668,.F.);
#82540=ORIENTED_EDGE('',*,*,#57393,.F.);
#82541=ORIENTED_EDGE('',*,*,#55498,.F.);
#82542=ORIENTED_EDGE('',*,*,#57392,.T.);
#82543=ORIENTED_EDGE('',*,*,#55501,.F.);
#82544=ORIENTED_EDGE('',*,*,#57394,.F.);
#82545=ORIENTED_EDGE('',*,*,#53659,.F.);
#82546=ORIENTED_EDGE('',*,*,#57393,.T.);
#82547=ORIENTED_EDGE('',*,*,#53686,.F.);
#82548=ORIENTED_EDGE('',*,*,#57395,.F.);
#82549=ORIENTED_EDGE('',*,*,#55499,.F.);
#82550=ORIENTED_EDGE('',*,*,#57394,.T.);
#82551=ORIENTED_EDGE('',*,*,#55500,.F.);
#82552=ORIENTED_EDGE('',*,*,#57395,.T.);
#82553=ORIENTED_EDGE('',*,*,#53664,.F.);
#82554=ORIENTED_EDGE('',*,*,#53660,.T.);
#82555=ORIENTED_EDGE('',*,*,#57396,.F.);
#82556=ORIENTED_EDGE('',*,*,#55540,.F.);
#82557=ORIENTED_EDGE('',*,*,#57397,.F.);
#82558=ORIENTED_EDGE('',*,*,#53616,.F.);
#82559=ORIENTED_EDGE('',*,*,#57397,.T.);
#82560=ORIENTED_EDGE('',*,*,#55539,.F.);
#82561=ORIENTED_EDGE('',*,*,#57398,.F.);
#82562=ORIENTED_EDGE('',*,*,#53625,.F.);
#82563=ORIENTED_EDGE('',*,*,#53615,.T.);
#82564=ORIENTED_EDGE('',*,*,#53619,.F.);
#82565=ORIENTED_EDGE('',*,*,#57399,.F.);
#82566=ORIENTED_EDGE('',*,*,#55541,.F.);
#82567=ORIENTED_EDGE('',*,*,#57396,.T.);
#82568=ORIENTED_EDGE('',*,*,#57398,.T.);
#82569=ORIENTED_EDGE('',*,*,#55538,.F.);
#82570=ORIENTED_EDGE('',*,*,#57400,.F.);
#82571=ORIENTED_EDGE('',*,*,#53610,.F.);
#82572=ORIENTED_EDGE('',*,*,#57399,.T.);
#82573=ORIENTED_EDGE('',*,*,#53623,.F.);
#82574=ORIENTED_EDGE('',*,*,#57401,.F.);
#82575=ORIENTED_EDGE('',*,*,#55530,.F.);
#82576=ORIENTED_EDGE('',*,*,#57400,.T.);
#82577=ORIENTED_EDGE('',*,*,#55537,.F.);
#82578=ORIENTED_EDGE('',*,*,#57402,.F.);
#82579=ORIENTED_EDGE('',*,*,#53627,.F.);
#82580=ORIENTED_EDGE('',*,*,#57401,.T.);
#82581=ORIENTED_EDGE('',*,*,#52258,.F.);
#82582=ORIENTED_EDGE('',*,*,#57403,.F.);
#82583=ORIENTED_EDGE('',*,*,#55531,.F.);
#82584=ORIENTED_EDGE('',*,*,#57402,.T.);
#82585=ORIENTED_EDGE('',*,*,#55536,.F.);
#82586=ORIENTED_EDGE('',*,*,#57404,.F.);
#82587=ORIENTED_EDGE('',*,*,#53602,.T.);
#82588=ORIENTED_EDGE('',*,*,#53606,.F.);
#82589=ORIENTED_EDGE('',*,*,#57403,.T.);
#82590=ORIENTED_EDGE('',*,*,#52257,.F.);
#82591=ORIENTED_EDGE('',*,*,#57405,.F.);
#82592=ORIENTED_EDGE('',*,*,#56420,.F.);
#82593=ORIENTED_EDGE('',*,*,#57404,.T.);
#82594=ORIENTED_EDGE('',*,*,#55535,.F.);
#82595=ORIENTED_EDGE('',*,*,#57406,.F.);
#82596=ORIENTED_EDGE('',*,*,#53603,.F.);
#82597=ORIENTED_EDGE('',*,*,#57405,.T.);
#82598=ORIENTED_EDGE('',*,*,#52256,.F.);
#82599=ORIENTED_EDGE('',*,*,#57407,.F.);
#82600=ORIENTED_EDGE('',*,*,#55515,.F.);
#82601=ORIENTED_EDGE('',*,*,#57406,.T.);
#82602=ORIENTED_EDGE('',*,*,#55534,.F.);
#82603=ORIENTED_EDGE('',*,*,#57408,.F.);
#82604=ORIENTED_EDGE('',*,*,#53621,.F.);
#82605=ORIENTED_EDGE('',*,*,#57407,.T.);
#82606=ORIENTED_EDGE('',*,*,#52255,.F.);
#82607=ORIENTED_EDGE('',*,*,#57409,.F.);
#82608=ORIENTED_EDGE('',*,*,#56422,.F.);
#82609=ORIENTED_EDGE('',*,*,#57408,.T.);
#82610=ORIENTED_EDGE('',*,*,#55533,.F.);
#82611=ORIENTED_EDGE('',*,*,#57410,.F.);
#82612=ORIENTED_EDGE('',*,*,#52769,.F.);
#82613=ORIENTED_EDGE('',*,*,#57409,.T.);
#82614=ORIENTED_EDGE('',*,*,#52254,.F.);
#82615=ORIENTED_EDGE('',*,*,#57411,.F.);
#82616=ORIENTED_EDGE('',*,*,#55521,.F.);
#82617=ORIENTED_EDGE('',*,*,#57410,.T.);
#82618=ORIENTED_EDGE('',*,*,#56421,.F.);
#82619=ORIENTED_EDGE('',*,*,#57412,.F.);
#82620=ORIENTED_EDGE('',*,*,#52770,.F.);
#82621=ORIENTED_EDGE('',*,*,#57411,.T.);
#82622=ORIENTED_EDGE('',*,*,#53652,.F.);
#82623=ORIENTED_EDGE('',*,*,#57413,.F.);
#82624=ORIENTED_EDGE('',*,*,#55522,.F.);
#82625=ORIENTED_EDGE('',*,*,#57412,.T.);
#82626=ORIENTED_EDGE('',*,*,#55517,.F.);
#82627=ORIENTED_EDGE('',*,*,#57414,.F.);
#82628=ORIENTED_EDGE('',*,*,#52771,.F.);
#82629=ORIENTED_EDGE('',*,*,#53647,.F.);
#82630=ORIENTED_EDGE('',*,*,#53643,.T.);
#82631=ORIENTED_EDGE('',*,*,#57415,.F.);
#82632=ORIENTED_EDGE('',*,*,#55523,.F.);
#82633=ORIENTED_EDGE('',*,*,#57413,.T.);
#82634=ORIENTED_EDGE('',*,*,#57414,.T.);
#82635=ORIENTED_EDGE('',*,*,#56423,.F.);
#82636=ORIENTED_EDGE('',*,*,#57416,.F.);
#82637=ORIENTED_EDGE('',*,*,#52772,.F.);
#82638=ORIENTED_EDGE('',*,*,#57415,.T.);
#82639=ORIENTED_EDGE('',*,*,#53642,.F.);
#82640=ORIENTED_EDGE('',*,*,#57417,.F.);
#82641=ORIENTED_EDGE('',*,*,#55524,.F.);
#82642=ORIENTED_EDGE('',*,*,#57416,.T.);
#82643=ORIENTED_EDGE('',*,*,#55519,.F.);
#82644=ORIENTED_EDGE('',*,*,#57418,.F.);
#82645=ORIENTED_EDGE('',*,*,#52773,.F.);
#82646=ORIENTED_EDGE('',*,*,#57417,.T.);
#82647=ORIENTED_EDGE('',*,*,#53654,.F.);
#82648=ORIENTED_EDGE('',*,*,#57419,.F.);
#82649=ORIENTED_EDGE('',*,*,#55525,.F.);
#82650=ORIENTED_EDGE('',*,*,#57418,.T.);
#82651=ORIENTED_EDGE('',*,*,#55518,.F.);
#82652=ORIENTED_EDGE('',*,*,#57420,.F.);
#82653=ORIENTED_EDGE('',*,*,#53650,.F.);
#82654=ORIENTED_EDGE('',*,*,#57419,.T.);
#82655=ORIENTED_EDGE('',*,*,#53638,.F.);
#82656=ORIENTED_EDGE('',*,*,#57421,.F.);
#82657=ORIENTED_EDGE('',*,*,#55526,.F.);
#82658=ORIENTED_EDGE('',*,*,#57420,.T.);
#82659=ORIENTED_EDGE('',*,*,#55529,.F.);
#82660=ORIENTED_EDGE('',*,*,#57422,.F.);
#82661=ORIENTED_EDGE('',*,*,#53629,.F.);
#82662=ORIENTED_EDGE('',*,*,#57421,.T.);
#82663=ORIENTED_EDGE('',*,*,#53656,.F.);
#82664=ORIENTED_EDGE('',*,*,#57423,.F.);
#82665=ORIENTED_EDGE('',*,*,#55527,.F.);
#82666=ORIENTED_EDGE('',*,*,#57422,.T.);
#82667=ORIENTED_EDGE('',*,*,#55528,.F.);
#82668=ORIENTED_EDGE('',*,*,#57423,.T.);
#82669=ORIENTED_EDGE('',*,*,#53634,.F.);
#82670=ORIENTED_EDGE('',*,*,#53630,.T.);
#82671=ORIENTED_EDGE('',*,*,#57424,.F.);
#82672=ORIENTED_EDGE('',*,*,#55568,.F.);
#82673=ORIENTED_EDGE('',*,*,#57425,.F.);
#82674=ORIENTED_EDGE('',*,*,#53586,.F.);
#82675=ORIENTED_EDGE('',*,*,#57425,.T.);
#82676=ORIENTED_EDGE('',*,*,#55567,.F.);
#82677=ORIENTED_EDGE('',*,*,#57426,.F.);
#82678=ORIENTED_EDGE('',*,*,#53595,.F.);
#82679=ORIENTED_EDGE('',*,*,#53585,.T.);
#82680=ORIENTED_EDGE('',*,*,#53589,.F.);
#82681=ORIENTED_EDGE('',*,*,#57427,.F.);
#82682=ORIENTED_EDGE('',*,*,#55569,.F.);
#82683=ORIENTED_EDGE('',*,*,#57424,.T.);
#82684=ORIENTED_EDGE('',*,*,#57426,.T.);
#82685=ORIENTED_EDGE('',*,*,#55566,.F.);
#82686=ORIENTED_EDGE('',*,*,#57428,.F.);
#82687=ORIENTED_EDGE('',*,*,#53580,.F.);
#82688=ORIENTED_EDGE('',*,*,#57427,.T.);
#82689=ORIENTED_EDGE('',*,*,#53593,.F.);
#82690=ORIENTED_EDGE('',*,*,#57429,.F.);
#82691=ORIENTED_EDGE('',*,*,#55558,.F.);
#82692=ORIENTED_EDGE('',*,*,#57428,.T.);
#82693=ORIENTED_EDGE('',*,*,#55565,.F.);
#82694=ORIENTED_EDGE('',*,*,#57430,.F.);
#82695=ORIENTED_EDGE('',*,*,#53597,.F.);
#82696=ORIENTED_EDGE('',*,*,#57429,.T.);
#82697=ORIENTED_EDGE('',*,*,#52264,.F.);
#82698=ORIENTED_EDGE('',*,*,#57431,.F.);
#82699=ORIENTED_EDGE('',*,*,#55559,.F.);
#82700=ORIENTED_EDGE('',*,*,#57430,.T.);
#82701=ORIENTED_EDGE('',*,*,#55564,.F.);
#82702=ORIENTED_EDGE('',*,*,#57432,.F.);
#82703=ORIENTED_EDGE('',*,*,#53572,.T.);
#82704=ORIENTED_EDGE('',*,*,#53576,.F.);
#82705=ORIENTED_EDGE('',*,*,#57431,.T.);
#82706=ORIENTED_EDGE('',*,*,#52263,.F.);
#82707=ORIENTED_EDGE('',*,*,#57433,.F.);
#82708=ORIENTED_EDGE('',*,*,#56424,.F.);
#82709=ORIENTED_EDGE('',*,*,#57432,.T.);
#82710=ORIENTED_EDGE('',*,*,#55563,.F.);
#82711=ORIENTED_EDGE('',*,*,#57434,.F.);
#82712=ORIENTED_EDGE('',*,*,#53573,.F.);
#82713=ORIENTED_EDGE('',*,*,#57433,.T.);
#82714=ORIENTED_EDGE('',*,*,#52262,.F.);
#82715=ORIENTED_EDGE('',*,*,#57435,.F.);
#82716=ORIENTED_EDGE('',*,*,#55543,.F.);
#82717=ORIENTED_EDGE('',*,*,#57434,.T.);
#82718=ORIENTED_EDGE('',*,*,#55562,.F.);
#82719=ORIENTED_EDGE('',*,*,#57436,.F.);
#82720=ORIENTED_EDGE('',*,*,#53591,.F.);
#82721=ORIENTED_EDGE('',*,*,#57435,.T.);
#82722=ORIENTED_EDGE('',*,*,#52261,.F.);
#82723=ORIENTED_EDGE('',*,*,#57437,.F.);
#82724=ORIENTED_EDGE('',*,*,#56426,.F.);
#82725=ORIENTED_EDGE('',*,*,#57436,.T.);
#82726=ORIENTED_EDGE('',*,*,#55561,.F.);
#82727=ORIENTED_EDGE('',*,*,#57438,.F.);
#82728=ORIENTED_EDGE('',*,*,#52763,.F.);
#82729=ORIENTED_EDGE('',*,*,#57437,.T.);
#82730=ORIENTED_EDGE('',*,*,#52260,.F.);
#82731=ORIENTED_EDGE('',*,*,#57439,.F.);
#82732=ORIENTED_EDGE('',*,*,#55549,.F.);
#82733=ORIENTED_EDGE('',*,*,#57438,.T.);
#82734=ORIENTED_EDGE('',*,*,#56425,.F.);
#82735=ORIENTED_EDGE('',*,*,#57440,.F.);
#82736=ORIENTED_EDGE('',*,*,#52764,.F.);
#82737=ORIENTED_EDGE('',*,*,#57439,.T.);
#82738=ORIENTED_EDGE('',*,*,#53622,.F.);
#82739=ORIENTED_EDGE('',*,*,#57441,.F.);
#82740=ORIENTED_EDGE('',*,*,#55550,.F.);
#82741=ORIENTED_EDGE('',*,*,#57440,.T.);
#82742=ORIENTED_EDGE('',*,*,#55545,.F.);
#82743=ORIENTED_EDGE('',*,*,#57442,.F.);
#82744=ORIENTED_EDGE('',*,*,#52765,.F.);
#82745=ORIENTED_EDGE('',*,*,#53617,.F.);
#82746=ORIENTED_EDGE('',*,*,#53613,.T.);
#82747=ORIENTED_EDGE('',*,*,#57443,.F.);
#82748=ORIENTED_EDGE('',*,*,#55551,.F.);
#82749=ORIENTED_EDGE('',*,*,#57441,.T.);
#82750=ORIENTED_EDGE('',*,*,#57442,.T.);
#82751=ORIENTED_EDGE('',*,*,#56427,.F.);
#82752=ORIENTED_EDGE('',*,*,#57444,.F.);
#82753=ORIENTED_EDGE('',*,*,#52766,.F.);
#82754=ORIENTED_EDGE('',*,*,#57443,.T.);
#82755=ORIENTED_EDGE('',*,*,#53612,.F.);
#82756=ORIENTED_EDGE('',*,*,#57445,.F.);
#82757=ORIENTED_EDGE('',*,*,#55552,.F.);
#82758=ORIENTED_EDGE('',*,*,#57444,.T.);
#82759=ORIENTED_EDGE('',*,*,#55547,.F.);
#82760=ORIENTED_EDGE('',*,*,#57446,.F.);
#82761=ORIENTED_EDGE('',*,*,#52767,.F.);
#82762=ORIENTED_EDGE('',*,*,#57445,.T.);
#82763=ORIENTED_EDGE('',*,*,#53624,.F.);
#82764=ORIENTED_EDGE('',*,*,#57447,.F.);
#82765=ORIENTED_EDGE('',*,*,#55553,.F.);
#82766=ORIENTED_EDGE('',*,*,#57446,.T.);
#82767=ORIENTED_EDGE('',*,*,#55546,.F.);
#82768=ORIENTED_EDGE('',*,*,#57448,.F.);
#82769=ORIENTED_EDGE('',*,*,#53620,.F.);
#82770=ORIENTED_EDGE('',*,*,#57447,.T.);
#82771=ORIENTED_EDGE('',*,*,#53608,.F.);
#82772=ORIENTED_EDGE('',*,*,#57449,.F.);
#82773=ORIENTED_EDGE('',*,*,#55554,.F.);
#82774=ORIENTED_EDGE('',*,*,#57448,.T.);
#82775=ORIENTED_EDGE('',*,*,#55557,.F.);
#82776=ORIENTED_EDGE('',*,*,#57450,.F.);
#82777=ORIENTED_EDGE('',*,*,#53599,.F.);
#82778=ORIENTED_EDGE('',*,*,#57449,.T.);
#82779=ORIENTED_EDGE('',*,*,#53626,.F.);
#82780=ORIENTED_EDGE('',*,*,#57451,.F.);
#82781=ORIENTED_EDGE('',*,*,#55555,.F.);
#82782=ORIENTED_EDGE('',*,*,#57450,.T.);
#82783=ORIENTED_EDGE('',*,*,#55556,.F.);
#82784=ORIENTED_EDGE('',*,*,#57451,.T.);
#82785=ORIENTED_EDGE('',*,*,#53604,.F.);
#82786=ORIENTED_EDGE('',*,*,#53600,.T.);
#82787=ORIENTED_EDGE('',*,*,#57452,.F.);
#82788=ORIENTED_EDGE('',*,*,#55596,.F.);
#82789=ORIENTED_EDGE('',*,*,#57453,.F.);
#82790=ORIENTED_EDGE('',*,*,#53556,.F.);
#82791=ORIENTED_EDGE('',*,*,#57453,.T.);
#82792=ORIENTED_EDGE('',*,*,#55595,.F.);
#82793=ORIENTED_EDGE('',*,*,#57454,.F.);
#82794=ORIENTED_EDGE('',*,*,#53565,.F.);
#82795=ORIENTED_EDGE('',*,*,#53555,.T.);
#82796=ORIENTED_EDGE('',*,*,#53559,.F.);
#82797=ORIENTED_EDGE('',*,*,#57455,.F.);
#82798=ORIENTED_EDGE('',*,*,#55597,.F.);
#82799=ORIENTED_EDGE('',*,*,#57452,.T.);
#82800=ORIENTED_EDGE('',*,*,#57454,.T.);
#82801=ORIENTED_EDGE('',*,*,#55594,.F.);
#82802=ORIENTED_EDGE('',*,*,#57456,.F.);
#82803=ORIENTED_EDGE('',*,*,#53550,.F.);
#82804=ORIENTED_EDGE('',*,*,#57455,.T.);
#82805=ORIENTED_EDGE('',*,*,#53563,.F.);
#82806=ORIENTED_EDGE('',*,*,#57457,.F.);
#82807=ORIENTED_EDGE('',*,*,#55586,.F.);
#82808=ORIENTED_EDGE('',*,*,#57456,.T.);
#82809=ORIENTED_EDGE('',*,*,#55593,.F.);
#82810=ORIENTED_EDGE('',*,*,#57458,.F.);
#82811=ORIENTED_EDGE('',*,*,#53567,.F.);
#82812=ORIENTED_EDGE('',*,*,#57457,.T.);
#82813=ORIENTED_EDGE('',*,*,#52270,.F.);
#82814=ORIENTED_EDGE('',*,*,#57459,.F.);
#82815=ORIENTED_EDGE('',*,*,#55587,.F.);
#82816=ORIENTED_EDGE('',*,*,#57458,.T.);
#82817=ORIENTED_EDGE('',*,*,#55592,.F.);
#82818=ORIENTED_EDGE('',*,*,#57460,.F.);
#82819=ORIENTED_EDGE('',*,*,#53542,.T.);
#82820=ORIENTED_EDGE('',*,*,#53546,.F.);
#82821=ORIENTED_EDGE('',*,*,#57459,.T.);
#82822=ORIENTED_EDGE('',*,*,#52269,.F.);
#82823=ORIENTED_EDGE('',*,*,#57461,.F.);
#82824=ORIENTED_EDGE('',*,*,#56428,.F.);
#82825=ORIENTED_EDGE('',*,*,#57460,.T.);
#82826=ORIENTED_EDGE('',*,*,#55591,.F.);
#82827=ORIENTED_EDGE('',*,*,#57462,.F.);
#82828=ORIENTED_EDGE('',*,*,#53543,.F.);
#82829=ORIENTED_EDGE('',*,*,#57461,.T.);
#82830=ORIENTED_EDGE('',*,*,#52268,.F.);
#82831=ORIENTED_EDGE('',*,*,#57463,.F.);
#82832=ORIENTED_EDGE('',*,*,#55571,.F.);
#82833=ORIENTED_EDGE('',*,*,#57462,.T.);
#82834=ORIENTED_EDGE('',*,*,#55590,.F.);
#82835=ORIENTED_EDGE('',*,*,#57464,.F.);
#82836=ORIENTED_EDGE('',*,*,#53561,.F.);
#82837=ORIENTED_EDGE('',*,*,#57463,.T.);
#82838=ORIENTED_EDGE('',*,*,#52267,.F.);
#82839=ORIENTED_EDGE('',*,*,#57465,.F.);
#82840=ORIENTED_EDGE('',*,*,#56430,.F.);
#82841=ORIENTED_EDGE('',*,*,#57464,.T.);
#82842=ORIENTED_EDGE('',*,*,#55589,.F.);
#82843=ORIENTED_EDGE('',*,*,#57466,.F.);
#82844=ORIENTED_EDGE('',*,*,#52757,.F.);
#82845=ORIENTED_EDGE('',*,*,#57465,.T.);
#82846=ORIENTED_EDGE('',*,*,#52266,.F.);
#82847=ORIENTED_EDGE('',*,*,#57467,.F.);
#82848=ORIENTED_EDGE('',*,*,#55577,.F.);
#82849=ORIENTED_EDGE('',*,*,#57466,.T.);
#82850=ORIENTED_EDGE('',*,*,#56429,.F.);
#82851=ORIENTED_EDGE('',*,*,#57468,.F.);
#82852=ORIENTED_EDGE('',*,*,#52758,.F.);
#82853=ORIENTED_EDGE('',*,*,#57467,.T.);
#82854=ORIENTED_EDGE('',*,*,#53592,.F.);
#82855=ORIENTED_EDGE('',*,*,#57469,.F.);
#82856=ORIENTED_EDGE('',*,*,#55578,.F.);
#82857=ORIENTED_EDGE('',*,*,#57468,.T.);
#82858=ORIENTED_EDGE('',*,*,#55573,.F.);
#82859=ORIENTED_EDGE('',*,*,#57470,.F.);
#82860=ORIENTED_EDGE('',*,*,#52759,.F.);
#82861=ORIENTED_EDGE('',*,*,#53587,.F.);
#82862=ORIENTED_EDGE('',*,*,#53583,.T.);
#82863=ORIENTED_EDGE('',*,*,#57471,.F.);
#82864=ORIENTED_EDGE('',*,*,#55579,.F.);
#82865=ORIENTED_EDGE('',*,*,#57469,.T.);
#82866=ORIENTED_EDGE('',*,*,#57470,.T.);
#82867=ORIENTED_EDGE('',*,*,#56431,.F.);
#82868=ORIENTED_EDGE('',*,*,#57472,.F.);
#82869=ORIENTED_EDGE('',*,*,#52760,.F.);
#82870=ORIENTED_EDGE('',*,*,#57471,.T.);
#82871=ORIENTED_EDGE('',*,*,#53582,.F.);
#82872=ORIENTED_EDGE('',*,*,#57473,.F.);
#82873=ORIENTED_EDGE('',*,*,#55580,.F.);
#82874=ORIENTED_EDGE('',*,*,#57472,.T.);
#82875=ORIENTED_EDGE('',*,*,#55575,.F.);
#82876=ORIENTED_EDGE('',*,*,#57474,.F.);
#82877=ORIENTED_EDGE('',*,*,#52761,.F.);
#82878=ORIENTED_EDGE('',*,*,#57473,.T.);
#82879=ORIENTED_EDGE('',*,*,#53594,.F.);
#82880=ORIENTED_EDGE('',*,*,#57475,.F.);
#82881=ORIENTED_EDGE('',*,*,#55581,.F.);
#82882=ORIENTED_EDGE('',*,*,#57474,.T.);
#82883=ORIENTED_EDGE('',*,*,#55574,.F.);
#82884=ORIENTED_EDGE('',*,*,#57476,.F.);
#82885=ORIENTED_EDGE('',*,*,#53590,.F.);
#82886=ORIENTED_EDGE('',*,*,#57475,.T.);
#82887=ORIENTED_EDGE('',*,*,#53578,.F.);
#82888=ORIENTED_EDGE('',*,*,#57477,.F.);
#82889=ORIENTED_EDGE('',*,*,#55582,.F.);
#82890=ORIENTED_EDGE('',*,*,#57476,.T.);
#82891=ORIENTED_EDGE('',*,*,#55585,.F.);
#82892=ORIENTED_EDGE('',*,*,#57478,.F.);
#82893=ORIENTED_EDGE('',*,*,#53569,.F.);
#82894=ORIENTED_EDGE('',*,*,#57477,.T.);
#82895=ORIENTED_EDGE('',*,*,#53596,.F.);
#82896=ORIENTED_EDGE('',*,*,#57479,.F.);
#82897=ORIENTED_EDGE('',*,*,#55583,.F.);
#82898=ORIENTED_EDGE('',*,*,#57478,.T.);
#82899=ORIENTED_EDGE('',*,*,#55584,.F.);
#82900=ORIENTED_EDGE('',*,*,#57479,.T.);
#82901=ORIENTED_EDGE('',*,*,#53574,.F.);
#82902=ORIENTED_EDGE('',*,*,#53570,.T.);
#82903=ORIENTED_EDGE('',*,*,#57480,.F.);
#82904=ORIENTED_EDGE('',*,*,#55624,.F.);
#82905=ORIENTED_EDGE('',*,*,#57481,.F.);
#82906=ORIENTED_EDGE('',*,*,#53526,.F.);
#82907=ORIENTED_EDGE('',*,*,#57481,.T.);
#82908=ORIENTED_EDGE('',*,*,#55623,.F.);
#82909=ORIENTED_EDGE('',*,*,#57482,.F.);
#82910=ORIENTED_EDGE('',*,*,#53535,.F.);
#82911=ORIENTED_EDGE('',*,*,#53525,.T.);
#82912=ORIENTED_EDGE('',*,*,#53529,.F.);
#82913=ORIENTED_EDGE('',*,*,#57483,.F.);
#82914=ORIENTED_EDGE('',*,*,#55625,.F.);
#82915=ORIENTED_EDGE('',*,*,#57480,.T.);
#82916=ORIENTED_EDGE('',*,*,#57482,.T.);
#82917=ORIENTED_EDGE('',*,*,#55622,.F.);
#82918=ORIENTED_EDGE('',*,*,#57484,.F.);
#82919=ORIENTED_EDGE('',*,*,#53520,.F.);
#82920=ORIENTED_EDGE('',*,*,#57483,.T.);
#82921=ORIENTED_EDGE('',*,*,#53533,.F.);
#82922=ORIENTED_EDGE('',*,*,#57485,.F.);
#82923=ORIENTED_EDGE('',*,*,#55614,.F.);
#82924=ORIENTED_EDGE('',*,*,#57484,.T.);
#82925=ORIENTED_EDGE('',*,*,#55621,.F.);
#82926=ORIENTED_EDGE('',*,*,#57486,.F.);
#82927=ORIENTED_EDGE('',*,*,#53537,.F.);
#82928=ORIENTED_EDGE('',*,*,#57485,.T.);
#82929=ORIENTED_EDGE('',*,*,#52276,.F.);
#82930=ORIENTED_EDGE('',*,*,#57487,.F.);
#82931=ORIENTED_EDGE('',*,*,#55615,.F.);
#82932=ORIENTED_EDGE('',*,*,#57486,.T.);
#82933=ORIENTED_EDGE('',*,*,#55620,.F.);
#82934=ORIENTED_EDGE('',*,*,#57488,.F.);
#82935=ORIENTED_EDGE('',*,*,#53512,.T.);
#82936=ORIENTED_EDGE('',*,*,#53516,.F.);
#82937=ORIENTED_EDGE('',*,*,#57487,.T.);
#82938=ORIENTED_EDGE('',*,*,#52275,.F.);
#82939=ORIENTED_EDGE('',*,*,#57489,.F.);
#82940=ORIENTED_EDGE('',*,*,#56432,.F.);
#82941=ORIENTED_EDGE('',*,*,#57488,.T.);
#82942=ORIENTED_EDGE('',*,*,#55619,.F.);
#82943=ORIENTED_EDGE('',*,*,#57490,.F.);
#82944=ORIENTED_EDGE('',*,*,#53513,.F.);
#82945=ORIENTED_EDGE('',*,*,#57489,.T.);
#82946=ORIENTED_EDGE('',*,*,#52274,.F.);
#82947=ORIENTED_EDGE('',*,*,#57491,.F.);
#82948=ORIENTED_EDGE('',*,*,#55599,.F.);
#82949=ORIENTED_EDGE('',*,*,#57490,.T.);
#82950=ORIENTED_EDGE('',*,*,#55618,.F.);
#82951=ORIENTED_EDGE('',*,*,#57492,.F.);
#82952=ORIENTED_EDGE('',*,*,#53531,.F.);
#82953=ORIENTED_EDGE('',*,*,#57491,.T.);
#82954=ORIENTED_EDGE('',*,*,#52273,.F.);
#82955=ORIENTED_EDGE('',*,*,#57493,.F.);
#82956=ORIENTED_EDGE('',*,*,#56434,.F.);
#82957=ORIENTED_EDGE('',*,*,#57492,.T.);
#82958=ORIENTED_EDGE('',*,*,#55617,.F.);
#82959=ORIENTED_EDGE('',*,*,#57494,.F.);
#82960=ORIENTED_EDGE('',*,*,#52751,.F.);
#82961=ORIENTED_EDGE('',*,*,#57493,.T.);
#82962=ORIENTED_EDGE('',*,*,#52272,.F.);
#82963=ORIENTED_EDGE('',*,*,#57495,.F.);
#82964=ORIENTED_EDGE('',*,*,#55605,.F.);
#82965=ORIENTED_EDGE('',*,*,#57494,.T.);
#82966=ORIENTED_EDGE('',*,*,#56433,.F.);
#82967=ORIENTED_EDGE('',*,*,#57496,.F.);
#82968=ORIENTED_EDGE('',*,*,#52752,.F.);
#82969=ORIENTED_EDGE('',*,*,#57495,.T.);
#82970=ORIENTED_EDGE('',*,*,#53562,.F.);
#82971=ORIENTED_EDGE('',*,*,#57497,.F.);
#82972=ORIENTED_EDGE('',*,*,#55606,.F.);
#82973=ORIENTED_EDGE('',*,*,#57496,.T.);
#82974=ORIENTED_EDGE('',*,*,#55601,.F.);
#82975=ORIENTED_EDGE('',*,*,#57498,.F.);
#82976=ORIENTED_EDGE('',*,*,#52753,.F.);
#82977=ORIENTED_EDGE('',*,*,#53557,.F.);
#82978=ORIENTED_EDGE('',*,*,#53553,.T.);
#82979=ORIENTED_EDGE('',*,*,#57499,.F.);
#82980=ORIENTED_EDGE('',*,*,#55607,.F.);
#82981=ORIENTED_EDGE('',*,*,#57497,.T.);
#82982=ORIENTED_EDGE('',*,*,#57498,.T.);
#82983=ORIENTED_EDGE('',*,*,#56435,.F.);
#82984=ORIENTED_EDGE('',*,*,#57500,.F.);
#82985=ORIENTED_EDGE('',*,*,#52754,.F.);
#82986=ORIENTED_EDGE('',*,*,#57499,.T.);
#82987=ORIENTED_EDGE('',*,*,#53552,.F.);
#82988=ORIENTED_EDGE('',*,*,#57501,.F.);
#82989=ORIENTED_EDGE('',*,*,#55608,.F.);
#82990=ORIENTED_EDGE('',*,*,#57500,.T.);
#82991=ORIENTED_EDGE('',*,*,#55603,.F.);
#82992=ORIENTED_EDGE('',*,*,#57502,.F.);
#82993=ORIENTED_EDGE('',*,*,#52755,.F.);
#82994=ORIENTED_EDGE('',*,*,#57501,.T.);
#82995=ORIENTED_EDGE('',*,*,#53564,.F.);
#82996=ORIENTED_EDGE('',*,*,#57503,.F.);
#82997=ORIENTED_EDGE('',*,*,#55609,.F.);
#82998=ORIENTED_EDGE('',*,*,#57502,.T.);
#82999=ORIENTED_EDGE('',*,*,#55602,.F.);
#83000=ORIENTED_EDGE('',*,*,#57504,.F.);
#83001=ORIENTED_EDGE('',*,*,#53560,.F.);
#83002=ORIENTED_EDGE('',*,*,#57503,.T.);
#83003=ORIENTED_EDGE('',*,*,#53548,.F.);
#83004=ORIENTED_EDGE('',*,*,#57505,.F.);
#83005=ORIENTED_EDGE('',*,*,#55610,.F.);
#83006=ORIENTED_EDGE('',*,*,#57504,.T.);
#83007=ORIENTED_EDGE('',*,*,#55613,.F.);
#83008=ORIENTED_EDGE('',*,*,#57506,.F.);
#83009=ORIENTED_EDGE('',*,*,#53539,.F.);
#83010=ORIENTED_EDGE('',*,*,#57505,.T.);
#83011=ORIENTED_EDGE('',*,*,#53566,.F.);
#83012=ORIENTED_EDGE('',*,*,#57507,.F.);
#83013=ORIENTED_EDGE('',*,*,#55611,.F.);
#83014=ORIENTED_EDGE('',*,*,#57506,.T.);
#83015=ORIENTED_EDGE('',*,*,#55612,.F.);
#83016=ORIENTED_EDGE('',*,*,#57507,.T.);
#83017=ORIENTED_EDGE('',*,*,#53544,.F.);
#83018=ORIENTED_EDGE('',*,*,#53540,.T.);
#83019=ORIENTED_EDGE('',*,*,#57508,.F.);
#83020=ORIENTED_EDGE('',*,*,#55652,.F.);
#83021=ORIENTED_EDGE('',*,*,#57509,.F.);
#83022=ORIENTED_EDGE('',*,*,#53496,.F.);
#83023=ORIENTED_EDGE('',*,*,#57509,.T.);
#83024=ORIENTED_EDGE('',*,*,#55651,.F.);
#83025=ORIENTED_EDGE('',*,*,#57510,.F.);
#83026=ORIENTED_EDGE('',*,*,#53505,.F.);
#83027=ORIENTED_EDGE('',*,*,#53495,.T.);
#83028=ORIENTED_EDGE('',*,*,#53499,.F.);
#83029=ORIENTED_EDGE('',*,*,#57511,.F.);
#83030=ORIENTED_EDGE('',*,*,#55653,.F.);
#83031=ORIENTED_EDGE('',*,*,#57508,.T.);
#83032=ORIENTED_EDGE('',*,*,#57510,.T.);
#83033=ORIENTED_EDGE('',*,*,#55650,.F.);
#83034=ORIENTED_EDGE('',*,*,#57512,.F.);
#83035=ORIENTED_EDGE('',*,*,#53490,.F.);
#83036=ORIENTED_EDGE('',*,*,#57511,.T.);
#83037=ORIENTED_EDGE('',*,*,#53503,.F.);
#83038=ORIENTED_EDGE('',*,*,#57513,.F.);
#83039=ORIENTED_EDGE('',*,*,#55642,.F.);
#83040=ORIENTED_EDGE('',*,*,#57512,.T.);
#83041=ORIENTED_EDGE('',*,*,#55649,.F.);
#83042=ORIENTED_EDGE('',*,*,#57514,.F.);
#83043=ORIENTED_EDGE('',*,*,#53507,.F.);
#83044=ORIENTED_EDGE('',*,*,#57513,.T.);
#83045=ORIENTED_EDGE('',*,*,#52282,.F.);
#83046=ORIENTED_EDGE('',*,*,#57515,.F.);
#83047=ORIENTED_EDGE('',*,*,#55643,.F.);
#83048=ORIENTED_EDGE('',*,*,#57514,.T.);
#83049=ORIENTED_EDGE('',*,*,#55648,.F.);
#83050=ORIENTED_EDGE('',*,*,#57516,.F.);
#83051=ORIENTED_EDGE('',*,*,#53482,.T.);
#83052=ORIENTED_EDGE('',*,*,#53486,.F.);
#83053=ORIENTED_EDGE('',*,*,#57515,.T.);
#83054=ORIENTED_EDGE('',*,*,#52281,.F.);
#83055=ORIENTED_EDGE('',*,*,#57517,.F.);
#83056=ORIENTED_EDGE('',*,*,#56436,.F.);
#83057=ORIENTED_EDGE('',*,*,#57516,.T.);
#83058=ORIENTED_EDGE('',*,*,#55647,.F.);
#83059=ORIENTED_EDGE('',*,*,#57518,.F.);
#83060=ORIENTED_EDGE('',*,*,#53483,.F.);
#83061=ORIENTED_EDGE('',*,*,#57517,.T.);
#83062=ORIENTED_EDGE('',*,*,#52280,.F.);
#83063=ORIENTED_EDGE('',*,*,#57519,.F.);
#83064=ORIENTED_EDGE('',*,*,#55627,.F.);
#83065=ORIENTED_EDGE('',*,*,#57518,.T.);
#83066=ORIENTED_EDGE('',*,*,#55646,.F.);
#83067=ORIENTED_EDGE('',*,*,#57520,.F.);
#83068=ORIENTED_EDGE('',*,*,#53501,.F.);
#83069=ORIENTED_EDGE('',*,*,#57519,.T.);
#83070=ORIENTED_EDGE('',*,*,#52279,.F.);
#83071=ORIENTED_EDGE('',*,*,#57521,.F.);
#83072=ORIENTED_EDGE('',*,*,#56438,.F.);
#83073=ORIENTED_EDGE('',*,*,#57520,.T.);
#83074=ORIENTED_EDGE('',*,*,#55645,.F.);
#83075=ORIENTED_EDGE('',*,*,#57522,.F.);
#83076=ORIENTED_EDGE('',*,*,#52745,.F.);
#83077=ORIENTED_EDGE('',*,*,#57521,.T.);
#83078=ORIENTED_EDGE('',*,*,#52278,.F.);
#83079=ORIENTED_EDGE('',*,*,#57523,.F.);
#83080=ORIENTED_EDGE('',*,*,#55633,.F.);
#83081=ORIENTED_EDGE('',*,*,#57522,.T.);
#83082=ORIENTED_EDGE('',*,*,#56437,.F.);
#83083=ORIENTED_EDGE('',*,*,#57524,.F.);
#83084=ORIENTED_EDGE('',*,*,#52746,.F.);
#83085=ORIENTED_EDGE('',*,*,#57523,.T.);
#83086=ORIENTED_EDGE('',*,*,#53532,.F.);
#83087=ORIENTED_EDGE('',*,*,#57525,.F.);
#83088=ORIENTED_EDGE('',*,*,#55634,.F.);
#83089=ORIENTED_EDGE('',*,*,#57524,.T.);
#83090=ORIENTED_EDGE('',*,*,#55629,.F.);
#83091=ORIENTED_EDGE('',*,*,#57526,.F.);
#83092=ORIENTED_EDGE('',*,*,#52747,.F.);
#83093=ORIENTED_EDGE('',*,*,#53527,.F.);
#83094=ORIENTED_EDGE('',*,*,#53523,.T.);
#83095=ORIENTED_EDGE('',*,*,#57527,.F.);
#83096=ORIENTED_EDGE('',*,*,#55635,.F.);
#83097=ORIENTED_EDGE('',*,*,#57525,.T.);
#83098=ORIENTED_EDGE('',*,*,#57526,.T.);
#83099=ORIENTED_EDGE('',*,*,#56439,.F.);
#83100=ORIENTED_EDGE('',*,*,#57528,.F.);
#83101=ORIENTED_EDGE('',*,*,#52748,.F.);
#83102=ORIENTED_EDGE('',*,*,#57527,.T.);
#83103=ORIENTED_EDGE('',*,*,#53522,.F.);
#83104=ORIENTED_EDGE('',*,*,#57529,.F.);
#83105=ORIENTED_EDGE('',*,*,#55636,.F.);
#83106=ORIENTED_EDGE('',*,*,#57528,.T.);
#83107=ORIENTED_EDGE('',*,*,#55631,.F.);
#83108=ORIENTED_EDGE('',*,*,#57530,.F.);
#83109=ORIENTED_EDGE('',*,*,#52749,.F.);
#83110=ORIENTED_EDGE('',*,*,#57529,.T.);
#83111=ORIENTED_EDGE('',*,*,#53534,.F.);
#83112=ORIENTED_EDGE('',*,*,#57531,.F.);
#83113=ORIENTED_EDGE('',*,*,#55637,.F.);
#83114=ORIENTED_EDGE('',*,*,#57530,.T.);
#83115=ORIENTED_EDGE('',*,*,#55630,.F.);
#83116=ORIENTED_EDGE('',*,*,#57532,.F.);
#83117=ORIENTED_EDGE('',*,*,#53530,.F.);
#83118=ORIENTED_EDGE('',*,*,#57531,.T.);
#83119=ORIENTED_EDGE('',*,*,#53518,.F.);
#83120=ORIENTED_EDGE('',*,*,#57533,.F.);
#83121=ORIENTED_EDGE('',*,*,#55638,.F.);
#83122=ORIENTED_EDGE('',*,*,#57532,.T.);
#83123=ORIENTED_EDGE('',*,*,#55641,.F.);
#83124=ORIENTED_EDGE('',*,*,#57534,.F.);
#83125=ORIENTED_EDGE('',*,*,#53509,.F.);
#83126=ORIENTED_EDGE('',*,*,#57533,.T.);
#83127=ORIENTED_EDGE('',*,*,#53536,.F.);
#83128=ORIENTED_EDGE('',*,*,#57535,.F.);
#83129=ORIENTED_EDGE('',*,*,#55639,.F.);
#83130=ORIENTED_EDGE('',*,*,#57534,.T.);
#83131=ORIENTED_EDGE('',*,*,#55640,.F.);
#83132=ORIENTED_EDGE('',*,*,#57535,.T.);
#83133=ORIENTED_EDGE('',*,*,#53514,.F.);
#83134=ORIENTED_EDGE('',*,*,#53510,.T.);
#83135=ORIENTED_EDGE('',*,*,#57536,.F.);
#83136=ORIENTED_EDGE('',*,*,#55680,.F.);
#83137=ORIENTED_EDGE('',*,*,#57537,.F.);
#83138=ORIENTED_EDGE('',*,*,#53466,.F.);
#83139=ORIENTED_EDGE('',*,*,#57537,.T.);
#83140=ORIENTED_EDGE('',*,*,#55679,.F.);
#83141=ORIENTED_EDGE('',*,*,#57538,.F.);
#83142=ORIENTED_EDGE('',*,*,#53475,.F.);
#83143=ORIENTED_EDGE('',*,*,#53465,.T.);
#83144=ORIENTED_EDGE('',*,*,#53469,.F.);
#83145=ORIENTED_EDGE('',*,*,#57539,.F.);
#83146=ORIENTED_EDGE('',*,*,#55681,.F.);
#83147=ORIENTED_EDGE('',*,*,#57536,.T.);
#83148=ORIENTED_EDGE('',*,*,#57538,.T.);
#83149=ORIENTED_EDGE('',*,*,#55678,.F.);
#83150=ORIENTED_EDGE('',*,*,#57540,.F.);
#83151=ORIENTED_EDGE('',*,*,#53460,.F.);
#83152=ORIENTED_EDGE('',*,*,#57539,.T.);
#83153=ORIENTED_EDGE('',*,*,#53473,.F.);
#83154=ORIENTED_EDGE('',*,*,#57541,.F.);
#83155=ORIENTED_EDGE('',*,*,#55670,.F.);
#83156=ORIENTED_EDGE('',*,*,#57540,.T.);
#83157=ORIENTED_EDGE('',*,*,#55677,.F.);
#83158=ORIENTED_EDGE('',*,*,#57542,.F.);
#83159=ORIENTED_EDGE('',*,*,#53477,.F.);
#83160=ORIENTED_EDGE('',*,*,#57541,.T.);
#83161=ORIENTED_EDGE('',*,*,#52288,.F.);
#83162=ORIENTED_EDGE('',*,*,#57543,.F.);
#83163=ORIENTED_EDGE('',*,*,#55671,.F.);
#83164=ORIENTED_EDGE('',*,*,#57542,.T.);
#83165=ORIENTED_EDGE('',*,*,#55676,.F.);
#83166=ORIENTED_EDGE('',*,*,#57544,.F.);
#83167=ORIENTED_EDGE('',*,*,#53452,.T.);
#83168=ORIENTED_EDGE('',*,*,#53456,.F.);
#83169=ORIENTED_EDGE('',*,*,#57543,.T.);
#83170=ORIENTED_EDGE('',*,*,#52287,.F.);
#83171=ORIENTED_EDGE('',*,*,#57545,.F.);
#83172=ORIENTED_EDGE('',*,*,#56440,.F.);
#83173=ORIENTED_EDGE('',*,*,#57544,.T.);
#83174=ORIENTED_EDGE('',*,*,#55675,.F.);
#83175=ORIENTED_EDGE('',*,*,#57546,.F.);
#83176=ORIENTED_EDGE('',*,*,#53453,.F.);
#83177=ORIENTED_EDGE('',*,*,#57545,.T.);
#83178=ORIENTED_EDGE('',*,*,#52286,.F.);
#83179=ORIENTED_EDGE('',*,*,#57547,.F.);
#83180=ORIENTED_EDGE('',*,*,#55655,.F.);
#83181=ORIENTED_EDGE('',*,*,#57546,.T.);
#83182=ORIENTED_EDGE('',*,*,#55674,.F.);
#83183=ORIENTED_EDGE('',*,*,#57548,.F.);
#83184=ORIENTED_EDGE('',*,*,#53471,.F.);
#83185=ORIENTED_EDGE('',*,*,#57547,.T.);
#83186=ORIENTED_EDGE('',*,*,#52285,.F.);
#83187=ORIENTED_EDGE('',*,*,#57549,.F.);
#83188=ORIENTED_EDGE('',*,*,#56442,.F.);
#83189=ORIENTED_EDGE('',*,*,#57548,.T.);
#83190=ORIENTED_EDGE('',*,*,#55673,.F.);
#83191=ORIENTED_EDGE('',*,*,#57550,.F.);
#83192=ORIENTED_EDGE('',*,*,#52739,.F.);
#83193=ORIENTED_EDGE('',*,*,#57549,.T.);
#83194=ORIENTED_EDGE('',*,*,#52284,.F.);
#83195=ORIENTED_EDGE('',*,*,#57551,.F.);
#83196=ORIENTED_EDGE('',*,*,#55661,.F.);
#83197=ORIENTED_EDGE('',*,*,#57550,.T.);
#83198=ORIENTED_EDGE('',*,*,#56441,.F.);
#83199=ORIENTED_EDGE('',*,*,#57552,.F.);
#83200=ORIENTED_EDGE('',*,*,#52740,.F.);
#83201=ORIENTED_EDGE('',*,*,#57551,.T.);
#83202=ORIENTED_EDGE('',*,*,#53502,.F.);
#83203=ORIENTED_EDGE('',*,*,#57553,.F.);
#83204=ORIENTED_EDGE('',*,*,#55662,.F.);
#83205=ORIENTED_EDGE('',*,*,#57552,.T.);
#83206=ORIENTED_EDGE('',*,*,#55657,.F.);
#83207=ORIENTED_EDGE('',*,*,#57554,.F.);
#83208=ORIENTED_EDGE('',*,*,#52741,.F.);
#83209=ORIENTED_EDGE('',*,*,#53497,.F.);
#83210=ORIENTED_EDGE('',*,*,#53493,.T.);
#83211=ORIENTED_EDGE('',*,*,#57555,.F.);
#83212=ORIENTED_EDGE('',*,*,#55663,.F.);
#83213=ORIENTED_EDGE('',*,*,#57553,.T.);
#83214=ORIENTED_EDGE('',*,*,#57554,.T.);
#83215=ORIENTED_EDGE('',*,*,#56443,.F.);
#83216=ORIENTED_EDGE('',*,*,#57556,.F.);
#83217=ORIENTED_EDGE('',*,*,#52742,.F.);
#83218=ORIENTED_EDGE('',*,*,#57555,.T.);
#83219=ORIENTED_EDGE('',*,*,#53492,.F.);
#83220=ORIENTED_EDGE('',*,*,#57557,.F.);
#83221=ORIENTED_EDGE('',*,*,#55664,.F.);
#83222=ORIENTED_EDGE('',*,*,#57556,.T.);
#83223=ORIENTED_EDGE('',*,*,#55659,.F.);
#83224=ORIENTED_EDGE('',*,*,#57558,.F.);
#83225=ORIENTED_EDGE('',*,*,#52743,.F.);
#83226=ORIENTED_EDGE('',*,*,#57557,.T.);
#83227=ORIENTED_EDGE('',*,*,#53504,.F.);
#83228=ORIENTED_EDGE('',*,*,#57559,.F.);
#83229=ORIENTED_EDGE('',*,*,#55665,.F.);
#83230=ORIENTED_EDGE('',*,*,#57558,.T.);
#83231=ORIENTED_EDGE('',*,*,#55658,.F.);
#83232=ORIENTED_EDGE('',*,*,#57560,.F.);
#83233=ORIENTED_EDGE('',*,*,#53500,.F.);
#83234=ORIENTED_EDGE('',*,*,#57559,.T.);
#83235=ORIENTED_EDGE('',*,*,#53488,.F.);
#83236=ORIENTED_EDGE('',*,*,#57561,.F.);
#83237=ORIENTED_EDGE('',*,*,#55666,.F.);
#83238=ORIENTED_EDGE('',*,*,#57560,.T.);
#83239=ORIENTED_EDGE('',*,*,#55669,.F.);
#83240=ORIENTED_EDGE('',*,*,#57562,.F.);
#83241=ORIENTED_EDGE('',*,*,#53479,.F.);
#83242=ORIENTED_EDGE('',*,*,#57561,.T.);
#83243=ORIENTED_EDGE('',*,*,#53506,.F.);
#83244=ORIENTED_EDGE('',*,*,#57563,.F.);
#83245=ORIENTED_EDGE('',*,*,#55667,.F.);
#83246=ORIENTED_EDGE('',*,*,#57562,.T.);
#83247=ORIENTED_EDGE('',*,*,#55668,.F.);
#83248=ORIENTED_EDGE('',*,*,#57563,.T.);
#83249=ORIENTED_EDGE('',*,*,#53484,.F.);
#83250=ORIENTED_EDGE('',*,*,#53480,.T.);
#83251=ORIENTED_EDGE('',*,*,#57564,.F.);
#83252=ORIENTED_EDGE('',*,*,#55708,.F.);
#83253=ORIENTED_EDGE('',*,*,#57565,.F.);
#83254=ORIENTED_EDGE('',*,*,#53436,.F.);
#83255=ORIENTED_EDGE('',*,*,#57565,.T.);
#83256=ORIENTED_EDGE('',*,*,#55707,.F.);
#83257=ORIENTED_EDGE('',*,*,#57566,.F.);
#83258=ORIENTED_EDGE('',*,*,#53445,.F.);
#83259=ORIENTED_EDGE('',*,*,#53435,.T.);
#83260=ORIENTED_EDGE('',*,*,#53439,.F.);
#83261=ORIENTED_EDGE('',*,*,#57567,.F.);
#83262=ORIENTED_EDGE('',*,*,#55709,.F.);
#83263=ORIENTED_EDGE('',*,*,#57564,.T.);
#83264=ORIENTED_EDGE('',*,*,#57566,.T.);
#83265=ORIENTED_EDGE('',*,*,#55706,.F.);
#83266=ORIENTED_EDGE('',*,*,#57568,.F.);
#83267=ORIENTED_EDGE('',*,*,#53430,.F.);
#83268=ORIENTED_EDGE('',*,*,#57567,.T.);
#83269=ORIENTED_EDGE('',*,*,#53443,.F.);
#83270=ORIENTED_EDGE('',*,*,#57569,.F.);
#83271=ORIENTED_EDGE('',*,*,#55698,.F.);
#83272=ORIENTED_EDGE('',*,*,#57568,.T.);
#83273=ORIENTED_EDGE('',*,*,#55705,.F.);
#83274=ORIENTED_EDGE('',*,*,#57570,.F.);
#83275=ORIENTED_EDGE('',*,*,#53447,.F.);
#83276=ORIENTED_EDGE('',*,*,#57569,.T.);
#83277=ORIENTED_EDGE('',*,*,#52294,.F.);
#83278=ORIENTED_EDGE('',*,*,#57571,.F.);
#83279=ORIENTED_EDGE('',*,*,#55699,.F.);
#83280=ORIENTED_EDGE('',*,*,#57570,.T.);
#83281=ORIENTED_EDGE('',*,*,#55704,.F.);
#83282=ORIENTED_EDGE('',*,*,#57572,.F.);
#83283=ORIENTED_EDGE('',*,*,#53422,.T.);
#83284=ORIENTED_EDGE('',*,*,#53426,.F.);
#83285=ORIENTED_EDGE('',*,*,#57571,.T.);
#83286=ORIENTED_EDGE('',*,*,#52293,.F.);
#83287=ORIENTED_EDGE('',*,*,#57573,.F.);
#83288=ORIENTED_EDGE('',*,*,#56444,.F.);
#83289=ORIENTED_EDGE('',*,*,#57572,.T.);
#83290=ORIENTED_EDGE('',*,*,#55703,.F.);
#83291=ORIENTED_EDGE('',*,*,#57574,.F.);
#83292=ORIENTED_EDGE('',*,*,#53423,.F.);
#83293=ORIENTED_EDGE('',*,*,#57573,.T.);
#83294=ORIENTED_EDGE('',*,*,#52292,.F.);
#83295=ORIENTED_EDGE('',*,*,#57575,.F.);
#83296=ORIENTED_EDGE('',*,*,#55683,.F.);
#83297=ORIENTED_EDGE('',*,*,#57574,.T.);
#83298=ORIENTED_EDGE('',*,*,#55702,.F.);
#83299=ORIENTED_EDGE('',*,*,#57576,.F.);
#83300=ORIENTED_EDGE('',*,*,#53441,.F.);
#83301=ORIENTED_EDGE('',*,*,#57575,.T.);
#83302=ORIENTED_EDGE('',*,*,#52291,.F.);
#83303=ORIENTED_EDGE('',*,*,#57577,.F.);
#83304=ORIENTED_EDGE('',*,*,#56446,.F.);
#83305=ORIENTED_EDGE('',*,*,#57576,.T.);
#83306=ORIENTED_EDGE('',*,*,#55701,.F.);
#83307=ORIENTED_EDGE('',*,*,#57578,.F.);
#83308=ORIENTED_EDGE('',*,*,#52733,.F.);
#83309=ORIENTED_EDGE('',*,*,#57577,.T.);
#83310=ORIENTED_EDGE('',*,*,#52290,.F.);
#83311=ORIENTED_EDGE('',*,*,#57579,.F.);
#83312=ORIENTED_EDGE('',*,*,#55689,.F.);
#83313=ORIENTED_EDGE('',*,*,#57578,.T.);
#83314=ORIENTED_EDGE('',*,*,#56445,.F.);
#83315=ORIENTED_EDGE('',*,*,#57580,.F.);
#83316=ORIENTED_EDGE('',*,*,#52734,.F.);
#83317=ORIENTED_EDGE('',*,*,#57579,.T.);
#83318=ORIENTED_EDGE('',*,*,#53472,.F.);
#83319=ORIENTED_EDGE('',*,*,#57581,.F.);
#83320=ORIENTED_EDGE('',*,*,#55690,.F.);
#83321=ORIENTED_EDGE('',*,*,#57580,.T.);
#83322=ORIENTED_EDGE('',*,*,#55685,.F.);
#83323=ORIENTED_EDGE('',*,*,#57582,.F.);
#83324=ORIENTED_EDGE('',*,*,#52735,.F.);
#83325=ORIENTED_EDGE('',*,*,#53467,.F.);
#83326=ORIENTED_EDGE('',*,*,#53463,.T.);
#83327=ORIENTED_EDGE('',*,*,#57583,.F.);
#83328=ORIENTED_EDGE('',*,*,#55691,.F.);
#83329=ORIENTED_EDGE('',*,*,#57581,.T.);
#83330=ORIENTED_EDGE('',*,*,#57582,.T.);
#83331=ORIENTED_EDGE('',*,*,#56447,.F.);
#83332=ORIENTED_EDGE('',*,*,#57584,.F.);
#83333=ORIENTED_EDGE('',*,*,#52736,.F.);
#83334=ORIENTED_EDGE('',*,*,#57583,.T.);
#83335=ORIENTED_EDGE('',*,*,#53462,.F.);
#83336=ORIENTED_EDGE('',*,*,#57585,.F.);
#83337=ORIENTED_EDGE('',*,*,#55692,.F.);
#83338=ORIENTED_EDGE('',*,*,#57584,.T.);
#83339=ORIENTED_EDGE('',*,*,#55687,.F.);
#83340=ORIENTED_EDGE('',*,*,#57586,.F.);
#83341=ORIENTED_EDGE('',*,*,#52737,.F.);
#83342=ORIENTED_EDGE('',*,*,#57585,.T.);
#83343=ORIENTED_EDGE('',*,*,#53474,.F.);
#83344=ORIENTED_EDGE('',*,*,#57587,.F.);
#83345=ORIENTED_EDGE('',*,*,#55693,.F.);
#83346=ORIENTED_EDGE('',*,*,#57586,.T.);
#83347=ORIENTED_EDGE('',*,*,#55686,.F.);
#83348=ORIENTED_EDGE('',*,*,#57588,.F.);
#83349=ORIENTED_EDGE('',*,*,#53470,.F.);
#83350=ORIENTED_EDGE('',*,*,#57587,.T.);
#83351=ORIENTED_EDGE('',*,*,#53458,.F.);
#83352=ORIENTED_EDGE('',*,*,#57589,.F.);
#83353=ORIENTED_EDGE('',*,*,#55694,.F.);
#83354=ORIENTED_EDGE('',*,*,#57588,.T.);
#83355=ORIENTED_EDGE('',*,*,#55697,.F.);
#83356=ORIENTED_EDGE('',*,*,#57590,.F.);
#83357=ORIENTED_EDGE('',*,*,#53449,.F.);
#83358=ORIENTED_EDGE('',*,*,#57589,.T.);
#83359=ORIENTED_EDGE('',*,*,#53476,.F.);
#83360=ORIENTED_EDGE('',*,*,#57591,.F.);
#83361=ORIENTED_EDGE('',*,*,#55695,.F.);
#83362=ORIENTED_EDGE('',*,*,#57590,.T.);
#83363=ORIENTED_EDGE('',*,*,#55696,.F.);
#83364=ORIENTED_EDGE('',*,*,#57591,.T.);
#83365=ORIENTED_EDGE('',*,*,#53454,.F.);
#83366=ORIENTED_EDGE('',*,*,#53450,.T.);
#83367=ORIENTED_EDGE('',*,*,#57592,.F.);
#83368=ORIENTED_EDGE('',*,*,#55736,.F.);
#83369=ORIENTED_EDGE('',*,*,#57593,.F.);
#83370=ORIENTED_EDGE('',*,*,#53406,.F.);
#83371=ORIENTED_EDGE('',*,*,#57593,.T.);
#83372=ORIENTED_EDGE('',*,*,#55735,.F.);
#83373=ORIENTED_EDGE('',*,*,#57594,.F.);
#83374=ORIENTED_EDGE('',*,*,#53415,.F.);
#83375=ORIENTED_EDGE('',*,*,#53405,.T.);
#83376=ORIENTED_EDGE('',*,*,#53409,.F.);
#83377=ORIENTED_EDGE('',*,*,#57595,.F.);
#83378=ORIENTED_EDGE('',*,*,#55737,.F.);
#83379=ORIENTED_EDGE('',*,*,#57592,.T.);
#83380=ORIENTED_EDGE('',*,*,#57594,.T.);
#83381=ORIENTED_EDGE('',*,*,#55734,.F.);
#83382=ORIENTED_EDGE('',*,*,#57596,.F.);
#83383=ORIENTED_EDGE('',*,*,#53400,.F.);
#83384=ORIENTED_EDGE('',*,*,#57595,.T.);
#83385=ORIENTED_EDGE('',*,*,#53413,.F.);
#83386=ORIENTED_EDGE('',*,*,#57597,.F.);
#83387=ORIENTED_EDGE('',*,*,#55726,.F.);
#83388=ORIENTED_EDGE('',*,*,#57596,.T.);
#83389=ORIENTED_EDGE('',*,*,#55733,.F.);
#83390=ORIENTED_EDGE('',*,*,#57598,.F.);
#83391=ORIENTED_EDGE('',*,*,#53417,.F.);
#83392=ORIENTED_EDGE('',*,*,#57597,.T.);
#83393=ORIENTED_EDGE('',*,*,#52300,.F.);
#83394=ORIENTED_EDGE('',*,*,#57599,.F.);
#83395=ORIENTED_EDGE('',*,*,#55727,.F.);
#83396=ORIENTED_EDGE('',*,*,#57598,.T.);
#83397=ORIENTED_EDGE('',*,*,#55732,.F.);
#83398=ORIENTED_EDGE('',*,*,#57600,.F.);
#83399=ORIENTED_EDGE('',*,*,#53392,.T.);
#83400=ORIENTED_EDGE('',*,*,#53396,.F.);
#83401=ORIENTED_EDGE('',*,*,#57599,.T.);
#83402=ORIENTED_EDGE('',*,*,#52299,.F.);
#83403=ORIENTED_EDGE('',*,*,#57601,.F.);
#83404=ORIENTED_EDGE('',*,*,#56448,.F.);
#83405=ORIENTED_EDGE('',*,*,#57600,.T.);
#83406=ORIENTED_EDGE('',*,*,#55731,.F.);
#83407=ORIENTED_EDGE('',*,*,#57602,.F.);
#83408=ORIENTED_EDGE('',*,*,#53393,.F.);
#83409=ORIENTED_EDGE('',*,*,#57601,.T.);
#83410=ORIENTED_EDGE('',*,*,#52298,.F.);
#83411=ORIENTED_EDGE('',*,*,#57603,.F.);
#83412=ORIENTED_EDGE('',*,*,#55711,.F.);
#83413=ORIENTED_EDGE('',*,*,#57602,.T.);
#83414=ORIENTED_EDGE('',*,*,#55730,.F.);
#83415=ORIENTED_EDGE('',*,*,#57604,.F.);
#83416=ORIENTED_EDGE('',*,*,#53411,.F.);
#83417=ORIENTED_EDGE('',*,*,#57603,.T.);
#83418=ORIENTED_EDGE('',*,*,#52297,.F.);
#83419=ORIENTED_EDGE('',*,*,#57605,.F.);
#83420=ORIENTED_EDGE('',*,*,#56450,.F.);
#83421=ORIENTED_EDGE('',*,*,#57604,.T.);
#83422=ORIENTED_EDGE('',*,*,#55729,.F.);
#83423=ORIENTED_EDGE('',*,*,#57606,.F.);
#83424=ORIENTED_EDGE('',*,*,#52727,.F.);
#83425=ORIENTED_EDGE('',*,*,#57605,.T.);
#83426=ORIENTED_EDGE('',*,*,#52296,.F.);
#83427=ORIENTED_EDGE('',*,*,#57607,.F.);
#83428=ORIENTED_EDGE('',*,*,#55717,.F.);
#83429=ORIENTED_EDGE('',*,*,#57606,.T.);
#83430=ORIENTED_EDGE('',*,*,#56449,.F.);
#83431=ORIENTED_EDGE('',*,*,#57608,.F.);
#83432=ORIENTED_EDGE('',*,*,#52728,.F.);
#83433=ORIENTED_EDGE('',*,*,#57607,.T.);
#83434=ORIENTED_EDGE('',*,*,#53442,.F.);
#83435=ORIENTED_EDGE('',*,*,#57609,.F.);
#83436=ORIENTED_EDGE('',*,*,#55718,.F.);
#83437=ORIENTED_EDGE('',*,*,#57608,.T.);
#83438=ORIENTED_EDGE('',*,*,#55713,.F.);
#83439=ORIENTED_EDGE('',*,*,#57610,.F.);
#83440=ORIENTED_EDGE('',*,*,#52729,.F.);
#83441=ORIENTED_EDGE('',*,*,#53437,.F.);
#83442=ORIENTED_EDGE('',*,*,#53433,.T.);
#83443=ORIENTED_EDGE('',*,*,#57611,.F.);
#83444=ORIENTED_EDGE('',*,*,#55719,.F.);
#83445=ORIENTED_EDGE('',*,*,#57609,.T.);
#83446=ORIENTED_EDGE('',*,*,#57610,.T.);
#83447=ORIENTED_EDGE('',*,*,#56451,.F.);
#83448=ORIENTED_EDGE('',*,*,#57612,.F.);
#83449=ORIENTED_EDGE('',*,*,#52730,.F.);
#83450=ORIENTED_EDGE('',*,*,#57611,.T.);
#83451=ORIENTED_EDGE('',*,*,#53432,.F.);
#83452=ORIENTED_EDGE('',*,*,#57613,.F.);
#83453=ORIENTED_EDGE('',*,*,#55720,.F.);
#83454=ORIENTED_EDGE('',*,*,#57612,.T.);
#83455=ORIENTED_EDGE('',*,*,#55715,.F.);
#83456=ORIENTED_EDGE('',*,*,#57614,.F.);
#83457=ORIENTED_EDGE('',*,*,#52731,.F.);
#83458=ORIENTED_EDGE('',*,*,#57613,.T.);
#83459=ORIENTED_EDGE('',*,*,#53444,.F.);
#83460=ORIENTED_EDGE('',*,*,#57615,.F.);
#83461=ORIENTED_EDGE('',*,*,#55721,.F.);
#83462=ORIENTED_EDGE('',*,*,#57614,.T.);
#83463=ORIENTED_EDGE('',*,*,#55714,.F.);
#83464=ORIENTED_EDGE('',*,*,#57616,.F.);
#83465=ORIENTED_EDGE('',*,*,#53440,.F.);
#83466=ORIENTED_EDGE('',*,*,#57615,.T.);
#83467=ORIENTED_EDGE('',*,*,#53428,.F.);
#83468=ORIENTED_EDGE('',*,*,#57617,.F.);
#83469=ORIENTED_EDGE('',*,*,#55722,.F.);
#83470=ORIENTED_EDGE('',*,*,#57616,.T.);
#83471=ORIENTED_EDGE('',*,*,#55725,.F.);
#83472=ORIENTED_EDGE('',*,*,#57618,.F.);
#83473=ORIENTED_EDGE('',*,*,#53419,.F.);
#83474=ORIENTED_EDGE('',*,*,#57617,.T.);
#83475=ORIENTED_EDGE('',*,*,#53446,.F.);
#83476=ORIENTED_EDGE('',*,*,#57619,.F.);
#83477=ORIENTED_EDGE('',*,*,#55723,.F.);
#83478=ORIENTED_EDGE('',*,*,#57618,.T.);
#83479=ORIENTED_EDGE('',*,*,#55724,.F.);
#83480=ORIENTED_EDGE('',*,*,#57619,.T.);
#83481=ORIENTED_EDGE('',*,*,#53424,.F.);
#83482=ORIENTED_EDGE('',*,*,#53420,.T.);
#83483=ORIENTED_EDGE('',*,*,#57620,.F.);
#83484=ORIENTED_EDGE('',*,*,#55764,.F.);
#83485=ORIENTED_EDGE('',*,*,#57621,.F.);
#83486=ORIENTED_EDGE('',*,*,#53376,.F.);
#83487=ORIENTED_EDGE('',*,*,#57621,.T.);
#83488=ORIENTED_EDGE('',*,*,#55763,.F.);
#83489=ORIENTED_EDGE('',*,*,#57622,.F.);
#83490=ORIENTED_EDGE('',*,*,#53385,.F.);
#83491=ORIENTED_EDGE('',*,*,#53375,.T.);
#83492=ORIENTED_EDGE('',*,*,#53379,.F.);
#83493=ORIENTED_EDGE('',*,*,#57623,.F.);
#83494=ORIENTED_EDGE('',*,*,#55765,.F.);
#83495=ORIENTED_EDGE('',*,*,#57620,.T.);
#83496=ORIENTED_EDGE('',*,*,#57622,.T.);
#83497=ORIENTED_EDGE('',*,*,#55762,.F.);
#83498=ORIENTED_EDGE('',*,*,#57624,.F.);
#83499=ORIENTED_EDGE('',*,*,#53370,.F.);
#83500=ORIENTED_EDGE('',*,*,#57623,.T.);
#83501=ORIENTED_EDGE('',*,*,#53383,.F.);
#83502=ORIENTED_EDGE('',*,*,#57625,.F.);
#83503=ORIENTED_EDGE('',*,*,#55754,.F.);
#83504=ORIENTED_EDGE('',*,*,#57624,.T.);
#83505=ORIENTED_EDGE('',*,*,#55761,.F.);
#83506=ORIENTED_EDGE('',*,*,#57626,.F.);
#83507=ORIENTED_EDGE('',*,*,#53387,.F.);
#83508=ORIENTED_EDGE('',*,*,#57625,.T.);
#83509=ORIENTED_EDGE('',*,*,#52306,.F.);
#83510=ORIENTED_EDGE('',*,*,#57627,.F.);
#83511=ORIENTED_EDGE('',*,*,#55755,.F.);
#83512=ORIENTED_EDGE('',*,*,#57626,.T.);
#83513=ORIENTED_EDGE('',*,*,#55760,.F.);
#83514=ORIENTED_EDGE('',*,*,#57628,.F.);
#83515=ORIENTED_EDGE('',*,*,#53362,.T.);
#83516=ORIENTED_EDGE('',*,*,#53366,.F.);
#83517=ORIENTED_EDGE('',*,*,#57627,.T.);
#83518=ORIENTED_EDGE('',*,*,#52305,.F.);
#83519=ORIENTED_EDGE('',*,*,#57629,.F.);
#83520=ORIENTED_EDGE('',*,*,#56452,.F.);
#83521=ORIENTED_EDGE('',*,*,#57628,.T.);
#83522=ORIENTED_EDGE('',*,*,#55759,.F.);
#83523=ORIENTED_EDGE('',*,*,#57630,.F.);
#83524=ORIENTED_EDGE('',*,*,#53363,.F.);
#83525=ORIENTED_EDGE('',*,*,#57629,.T.);
#83526=ORIENTED_EDGE('',*,*,#52304,.F.);
#83527=ORIENTED_EDGE('',*,*,#57631,.F.);
#83528=ORIENTED_EDGE('',*,*,#55739,.F.);
#83529=ORIENTED_EDGE('',*,*,#57630,.T.);
#83530=ORIENTED_EDGE('',*,*,#55758,.F.);
#83531=ORIENTED_EDGE('',*,*,#57632,.F.);
#83532=ORIENTED_EDGE('',*,*,#53381,.F.);
#83533=ORIENTED_EDGE('',*,*,#57631,.T.);
#83534=ORIENTED_EDGE('',*,*,#52303,.F.);
#83535=ORIENTED_EDGE('',*,*,#57633,.F.);
#83536=ORIENTED_EDGE('',*,*,#56454,.F.);
#83537=ORIENTED_EDGE('',*,*,#57632,.T.);
#83538=ORIENTED_EDGE('',*,*,#55757,.F.);
#83539=ORIENTED_EDGE('',*,*,#57634,.F.);
#83540=ORIENTED_EDGE('',*,*,#52721,.F.);
#83541=ORIENTED_EDGE('',*,*,#57633,.T.);
#83542=ORIENTED_EDGE('',*,*,#52302,.F.);
#83543=ORIENTED_EDGE('',*,*,#57635,.F.);
#83544=ORIENTED_EDGE('',*,*,#55745,.F.);
#83545=ORIENTED_EDGE('',*,*,#57634,.T.);
#83546=ORIENTED_EDGE('',*,*,#56453,.F.);
#83547=ORIENTED_EDGE('',*,*,#57636,.F.);
#83548=ORIENTED_EDGE('',*,*,#52722,.F.);
#83549=ORIENTED_EDGE('',*,*,#57635,.T.);
#83550=ORIENTED_EDGE('',*,*,#53412,.F.);
#83551=ORIENTED_EDGE('',*,*,#57637,.F.);
#83552=ORIENTED_EDGE('',*,*,#55746,.F.);
#83553=ORIENTED_EDGE('',*,*,#57636,.T.);
#83554=ORIENTED_EDGE('',*,*,#55741,.F.);
#83555=ORIENTED_EDGE('',*,*,#57638,.F.);
#83556=ORIENTED_EDGE('',*,*,#52723,.F.);
#83557=ORIENTED_EDGE('',*,*,#53407,.F.);
#83558=ORIENTED_EDGE('',*,*,#53403,.T.);
#83559=ORIENTED_EDGE('',*,*,#57639,.F.);
#83560=ORIENTED_EDGE('',*,*,#55747,.F.);
#83561=ORIENTED_EDGE('',*,*,#57637,.T.);
#83562=ORIENTED_EDGE('',*,*,#57638,.T.);
#83563=ORIENTED_EDGE('',*,*,#56455,.F.);
#83564=ORIENTED_EDGE('',*,*,#57640,.F.);
#83565=ORIENTED_EDGE('',*,*,#52724,.F.);
#83566=ORIENTED_EDGE('',*,*,#57639,.T.);
#83567=ORIENTED_EDGE('',*,*,#53402,.F.);
#83568=ORIENTED_EDGE('',*,*,#57641,.F.);
#83569=ORIENTED_EDGE('',*,*,#55748,.F.);
#83570=ORIENTED_EDGE('',*,*,#57640,.T.);
#83571=ORIENTED_EDGE('',*,*,#55743,.F.);
#83572=ORIENTED_EDGE('',*,*,#57642,.F.);
#83573=ORIENTED_EDGE('',*,*,#52725,.F.);
#83574=ORIENTED_EDGE('',*,*,#57641,.T.);
#83575=ORIENTED_EDGE('',*,*,#53414,.F.);
#83576=ORIENTED_EDGE('',*,*,#57643,.F.);
#83577=ORIENTED_EDGE('',*,*,#55749,.F.);
#83578=ORIENTED_EDGE('',*,*,#57642,.T.);
#83579=ORIENTED_EDGE('',*,*,#55742,.F.);
#83580=ORIENTED_EDGE('',*,*,#57644,.F.);
#83581=ORIENTED_EDGE('',*,*,#53410,.F.);
#83582=ORIENTED_EDGE('',*,*,#57643,.T.);
#83583=ORIENTED_EDGE('',*,*,#53398,.F.);
#83584=ORIENTED_EDGE('',*,*,#57645,.F.);
#83585=ORIENTED_EDGE('',*,*,#55750,.F.);
#83586=ORIENTED_EDGE('',*,*,#57644,.T.);
#83587=ORIENTED_EDGE('',*,*,#55753,.F.);
#83588=ORIENTED_EDGE('',*,*,#57646,.F.);
#83589=ORIENTED_EDGE('',*,*,#53389,.F.);
#83590=ORIENTED_EDGE('',*,*,#57645,.T.);
#83591=ORIENTED_EDGE('',*,*,#53416,.F.);
#83592=ORIENTED_EDGE('',*,*,#57647,.F.);
#83593=ORIENTED_EDGE('',*,*,#55751,.F.);
#83594=ORIENTED_EDGE('',*,*,#57646,.T.);
#83595=ORIENTED_EDGE('',*,*,#55752,.F.);
#83596=ORIENTED_EDGE('',*,*,#57647,.T.);
#83597=ORIENTED_EDGE('',*,*,#53394,.F.);
#83598=ORIENTED_EDGE('',*,*,#53390,.T.);
#83599=ORIENTED_EDGE('',*,*,#57648,.F.);
#83600=ORIENTED_EDGE('',*,*,#55792,.F.);
#83601=ORIENTED_EDGE('',*,*,#57649,.F.);
#83602=ORIENTED_EDGE('',*,*,#53346,.F.);
#83603=ORIENTED_EDGE('',*,*,#57649,.T.);
#83604=ORIENTED_EDGE('',*,*,#55791,.F.);
#83605=ORIENTED_EDGE('',*,*,#57650,.F.);
#83606=ORIENTED_EDGE('',*,*,#53355,.F.);
#83607=ORIENTED_EDGE('',*,*,#53345,.T.);
#83608=ORIENTED_EDGE('',*,*,#53349,.F.);
#83609=ORIENTED_EDGE('',*,*,#57651,.F.);
#83610=ORIENTED_EDGE('',*,*,#55793,.F.);
#83611=ORIENTED_EDGE('',*,*,#57648,.T.);
#83612=ORIENTED_EDGE('',*,*,#57650,.T.);
#83613=ORIENTED_EDGE('',*,*,#55790,.F.);
#83614=ORIENTED_EDGE('',*,*,#57652,.F.);
#83615=ORIENTED_EDGE('',*,*,#53340,.F.);
#83616=ORIENTED_EDGE('',*,*,#57651,.T.);
#83617=ORIENTED_EDGE('',*,*,#53353,.F.);
#83618=ORIENTED_EDGE('',*,*,#57653,.F.);
#83619=ORIENTED_EDGE('',*,*,#55782,.F.);
#83620=ORIENTED_EDGE('',*,*,#57652,.T.);
#83621=ORIENTED_EDGE('',*,*,#55789,.F.);
#83622=ORIENTED_EDGE('',*,*,#57654,.F.);
#83623=ORIENTED_EDGE('',*,*,#53357,.F.);
#83624=ORIENTED_EDGE('',*,*,#57653,.T.);
#83625=ORIENTED_EDGE('',*,*,#52312,.F.);
#83626=ORIENTED_EDGE('',*,*,#57655,.F.);
#83627=ORIENTED_EDGE('',*,*,#55783,.F.);
#83628=ORIENTED_EDGE('',*,*,#57654,.T.);
#83629=ORIENTED_EDGE('',*,*,#55788,.F.);
#83630=ORIENTED_EDGE('',*,*,#57656,.F.);
#83631=ORIENTED_EDGE('',*,*,#53332,.T.);
#83632=ORIENTED_EDGE('',*,*,#53336,.F.);
#83633=ORIENTED_EDGE('',*,*,#57655,.T.);
#83634=ORIENTED_EDGE('',*,*,#52311,.F.);
#83635=ORIENTED_EDGE('',*,*,#57657,.F.);
#83636=ORIENTED_EDGE('',*,*,#56456,.F.);
#83637=ORIENTED_EDGE('',*,*,#57656,.T.);
#83638=ORIENTED_EDGE('',*,*,#55787,.F.);
#83639=ORIENTED_EDGE('',*,*,#57658,.F.);
#83640=ORIENTED_EDGE('',*,*,#53333,.F.);
#83641=ORIENTED_EDGE('',*,*,#57657,.T.);
#83642=ORIENTED_EDGE('',*,*,#52310,.F.);
#83643=ORIENTED_EDGE('',*,*,#57659,.F.);
#83644=ORIENTED_EDGE('',*,*,#55767,.F.);
#83645=ORIENTED_EDGE('',*,*,#57658,.T.);
#83646=ORIENTED_EDGE('',*,*,#55786,.F.);
#83647=ORIENTED_EDGE('',*,*,#57660,.F.);
#83648=ORIENTED_EDGE('',*,*,#53351,.F.);
#83649=ORIENTED_EDGE('',*,*,#57659,.T.);
#83650=ORIENTED_EDGE('',*,*,#52309,.F.);
#83651=ORIENTED_EDGE('',*,*,#57661,.F.);
#83652=ORIENTED_EDGE('',*,*,#56458,.F.);
#83653=ORIENTED_EDGE('',*,*,#57660,.T.);
#83654=ORIENTED_EDGE('',*,*,#55785,.F.);
#83655=ORIENTED_EDGE('',*,*,#57662,.F.);
#83656=ORIENTED_EDGE('',*,*,#52715,.F.);
#83657=ORIENTED_EDGE('',*,*,#57661,.T.);
#83658=ORIENTED_EDGE('',*,*,#52308,.F.);
#83659=ORIENTED_EDGE('',*,*,#57663,.F.);
#83660=ORIENTED_EDGE('',*,*,#55773,.F.);
#83661=ORIENTED_EDGE('',*,*,#57662,.T.);
#83662=ORIENTED_EDGE('',*,*,#56457,.F.);
#83663=ORIENTED_EDGE('',*,*,#57664,.F.);
#83664=ORIENTED_EDGE('',*,*,#52716,.F.);
#83665=ORIENTED_EDGE('',*,*,#57663,.T.);
#83666=ORIENTED_EDGE('',*,*,#53382,.F.);
#83667=ORIENTED_EDGE('',*,*,#57665,.F.);
#83668=ORIENTED_EDGE('',*,*,#55774,.F.);
#83669=ORIENTED_EDGE('',*,*,#57664,.T.);
#83670=ORIENTED_EDGE('',*,*,#55769,.F.);
#83671=ORIENTED_EDGE('',*,*,#57666,.F.);
#83672=ORIENTED_EDGE('',*,*,#52717,.F.);
#83673=ORIENTED_EDGE('',*,*,#53377,.F.);
#83674=ORIENTED_EDGE('',*,*,#53373,.T.);
#83675=ORIENTED_EDGE('',*,*,#57667,.F.);
#83676=ORIENTED_EDGE('',*,*,#55775,.F.);
#83677=ORIENTED_EDGE('',*,*,#57665,.T.);
#83678=ORIENTED_EDGE('',*,*,#57666,.T.);
#83679=ORIENTED_EDGE('',*,*,#56459,.F.);
#83680=ORIENTED_EDGE('',*,*,#57668,.F.);
#83681=ORIENTED_EDGE('',*,*,#52718,.F.);
#83682=ORIENTED_EDGE('',*,*,#57667,.T.);
#83683=ORIENTED_EDGE('',*,*,#53372,.F.);
#83684=ORIENTED_EDGE('',*,*,#57669,.F.);
#83685=ORIENTED_EDGE('',*,*,#55776,.F.);
#83686=ORIENTED_EDGE('',*,*,#57668,.T.);
#83687=ORIENTED_EDGE('',*,*,#55771,.F.);
#83688=ORIENTED_EDGE('',*,*,#57670,.F.);
#83689=ORIENTED_EDGE('',*,*,#52719,.F.);
#83690=ORIENTED_EDGE('',*,*,#57669,.T.);
#83691=ORIENTED_EDGE('',*,*,#53384,.F.);
#83692=ORIENTED_EDGE('',*,*,#57671,.F.);
#83693=ORIENTED_EDGE('',*,*,#55777,.F.);
#83694=ORIENTED_EDGE('',*,*,#57670,.T.);
#83695=ORIENTED_EDGE('',*,*,#55770,.F.);
#83696=ORIENTED_EDGE('',*,*,#57672,.F.);
#83697=ORIENTED_EDGE('',*,*,#53380,.F.);
#83698=ORIENTED_EDGE('',*,*,#57671,.T.);
#83699=ORIENTED_EDGE('',*,*,#53368,.F.);
#83700=ORIENTED_EDGE('',*,*,#57673,.F.);
#83701=ORIENTED_EDGE('',*,*,#55778,.F.);
#83702=ORIENTED_EDGE('',*,*,#57672,.T.);
#83703=ORIENTED_EDGE('',*,*,#55781,.F.);
#83704=ORIENTED_EDGE('',*,*,#57674,.F.);
#83705=ORIENTED_EDGE('',*,*,#53359,.F.);
#83706=ORIENTED_EDGE('',*,*,#57673,.T.);
#83707=ORIENTED_EDGE('',*,*,#53386,.F.);
#83708=ORIENTED_EDGE('',*,*,#57675,.F.);
#83709=ORIENTED_EDGE('',*,*,#55779,.F.);
#83710=ORIENTED_EDGE('',*,*,#57674,.T.);
#83711=ORIENTED_EDGE('',*,*,#55780,.F.);
#83712=ORIENTED_EDGE('',*,*,#57675,.T.);
#83713=ORIENTED_EDGE('',*,*,#53364,.F.);
#83714=ORIENTED_EDGE('',*,*,#53360,.T.);
#83715=ORIENTED_EDGE('',*,*,#57676,.F.);
#83716=ORIENTED_EDGE('',*,*,#55820,.F.);
#83717=ORIENTED_EDGE('',*,*,#57677,.F.);
#83718=ORIENTED_EDGE('',*,*,#53316,.F.);
#83719=ORIENTED_EDGE('',*,*,#57677,.T.);
#83720=ORIENTED_EDGE('',*,*,#55819,.F.);
#83721=ORIENTED_EDGE('',*,*,#57678,.F.);
#83722=ORIENTED_EDGE('',*,*,#53325,.F.);
#83723=ORIENTED_EDGE('',*,*,#53315,.T.);
#83724=ORIENTED_EDGE('',*,*,#53319,.F.);
#83725=ORIENTED_EDGE('',*,*,#57679,.F.);
#83726=ORIENTED_EDGE('',*,*,#55821,.F.);
#83727=ORIENTED_EDGE('',*,*,#57676,.T.);
#83728=ORIENTED_EDGE('',*,*,#57678,.T.);
#83729=ORIENTED_EDGE('',*,*,#55818,.F.);
#83730=ORIENTED_EDGE('',*,*,#57680,.F.);
#83731=ORIENTED_EDGE('',*,*,#53310,.F.);
#83732=ORIENTED_EDGE('',*,*,#57679,.T.);
#83733=ORIENTED_EDGE('',*,*,#53323,.F.);
#83734=ORIENTED_EDGE('',*,*,#57681,.F.);
#83735=ORIENTED_EDGE('',*,*,#55810,.F.);
#83736=ORIENTED_EDGE('',*,*,#57680,.T.);
#83737=ORIENTED_EDGE('',*,*,#55817,.F.);
#83738=ORIENTED_EDGE('',*,*,#57682,.F.);
#83739=ORIENTED_EDGE('',*,*,#53327,.F.);
#83740=ORIENTED_EDGE('',*,*,#57681,.T.);
#83741=ORIENTED_EDGE('',*,*,#52318,.F.);
#83742=ORIENTED_EDGE('',*,*,#57683,.F.);
#83743=ORIENTED_EDGE('',*,*,#55811,.F.);
#83744=ORIENTED_EDGE('',*,*,#57682,.T.);
#83745=ORIENTED_EDGE('',*,*,#55816,.F.);
#83746=ORIENTED_EDGE('',*,*,#57684,.F.);
#83747=ORIENTED_EDGE('',*,*,#53302,.T.);
#83748=ORIENTED_EDGE('',*,*,#53306,.F.);
#83749=ORIENTED_EDGE('',*,*,#57683,.T.);
#83750=ORIENTED_EDGE('',*,*,#52317,.F.);
#83751=ORIENTED_EDGE('',*,*,#57685,.F.);
#83752=ORIENTED_EDGE('',*,*,#56460,.F.);
#83753=ORIENTED_EDGE('',*,*,#57684,.T.);
#83754=ORIENTED_EDGE('',*,*,#55815,.F.);
#83755=ORIENTED_EDGE('',*,*,#57686,.F.);
#83756=ORIENTED_EDGE('',*,*,#53303,.F.);
#83757=ORIENTED_EDGE('',*,*,#57685,.T.);
#83758=ORIENTED_EDGE('',*,*,#52316,.F.);
#83759=ORIENTED_EDGE('',*,*,#57687,.F.);
#83760=ORIENTED_EDGE('',*,*,#55795,.F.);
#83761=ORIENTED_EDGE('',*,*,#57686,.T.);
#83762=ORIENTED_EDGE('',*,*,#55814,.F.);
#83763=ORIENTED_EDGE('',*,*,#57688,.F.);
#83764=ORIENTED_EDGE('',*,*,#53321,.F.);
#83765=ORIENTED_EDGE('',*,*,#57687,.T.);
#83766=ORIENTED_EDGE('',*,*,#52315,.F.);
#83767=ORIENTED_EDGE('',*,*,#57689,.F.);
#83768=ORIENTED_EDGE('',*,*,#56462,.F.);
#83769=ORIENTED_EDGE('',*,*,#57688,.T.);
#83770=ORIENTED_EDGE('',*,*,#55813,.F.);
#83771=ORIENTED_EDGE('',*,*,#57690,.F.);
#83772=ORIENTED_EDGE('',*,*,#52709,.F.);
#83773=ORIENTED_EDGE('',*,*,#57689,.T.);
#83774=ORIENTED_EDGE('',*,*,#52314,.F.);
#83775=ORIENTED_EDGE('',*,*,#57691,.F.);
#83776=ORIENTED_EDGE('',*,*,#55801,.F.);
#83777=ORIENTED_EDGE('',*,*,#57690,.T.);
#83778=ORIENTED_EDGE('',*,*,#56461,.F.);
#83779=ORIENTED_EDGE('',*,*,#57692,.F.);
#83780=ORIENTED_EDGE('',*,*,#52710,.F.);
#83781=ORIENTED_EDGE('',*,*,#57691,.T.);
#83782=ORIENTED_EDGE('',*,*,#53352,.F.);
#83783=ORIENTED_EDGE('',*,*,#57693,.F.);
#83784=ORIENTED_EDGE('',*,*,#55802,.F.);
#83785=ORIENTED_EDGE('',*,*,#57692,.T.);
#83786=ORIENTED_EDGE('',*,*,#55797,.F.);
#83787=ORIENTED_EDGE('',*,*,#57694,.F.);
#83788=ORIENTED_EDGE('',*,*,#52711,.F.);
#83789=ORIENTED_EDGE('',*,*,#53347,.F.);
#83790=ORIENTED_EDGE('',*,*,#53343,.T.);
#83791=ORIENTED_EDGE('',*,*,#57695,.F.);
#83792=ORIENTED_EDGE('',*,*,#55803,.F.);
#83793=ORIENTED_EDGE('',*,*,#57693,.T.);
#83794=ORIENTED_EDGE('',*,*,#57694,.T.);
#83795=ORIENTED_EDGE('',*,*,#56463,.F.);
#83796=ORIENTED_EDGE('',*,*,#57696,.F.);
#83797=ORIENTED_EDGE('',*,*,#52712,.F.);
#83798=ORIENTED_EDGE('',*,*,#57695,.T.);
#83799=ORIENTED_EDGE('',*,*,#53342,.F.);
#83800=ORIENTED_EDGE('',*,*,#57697,.F.);
#83801=ORIENTED_EDGE('',*,*,#55804,.F.);
#83802=ORIENTED_EDGE('',*,*,#57696,.T.);
#83803=ORIENTED_EDGE('',*,*,#55799,.F.);
#83804=ORIENTED_EDGE('',*,*,#57698,.F.);
#83805=ORIENTED_EDGE('',*,*,#52713,.F.);
#83806=ORIENTED_EDGE('',*,*,#57697,.T.);
#83807=ORIENTED_EDGE('',*,*,#53354,.F.);
#83808=ORIENTED_EDGE('',*,*,#57699,.F.);
#83809=ORIENTED_EDGE('',*,*,#55805,.F.);
#83810=ORIENTED_EDGE('',*,*,#57698,.T.);
#83811=ORIENTED_EDGE('',*,*,#55798,.F.);
#83812=ORIENTED_EDGE('',*,*,#57700,.F.);
#83813=ORIENTED_EDGE('',*,*,#53350,.F.);
#83814=ORIENTED_EDGE('',*,*,#57699,.T.);
#83815=ORIENTED_EDGE('',*,*,#53338,.F.);
#83816=ORIENTED_EDGE('',*,*,#57701,.F.);
#83817=ORIENTED_EDGE('',*,*,#55806,.F.);
#83818=ORIENTED_EDGE('',*,*,#57700,.T.);
#83819=ORIENTED_EDGE('',*,*,#55809,.F.);
#83820=ORIENTED_EDGE('',*,*,#57702,.F.);
#83821=ORIENTED_EDGE('',*,*,#53329,.F.);
#83822=ORIENTED_EDGE('',*,*,#57701,.T.);
#83823=ORIENTED_EDGE('',*,*,#53356,.F.);
#83824=ORIENTED_EDGE('',*,*,#57703,.F.);
#83825=ORIENTED_EDGE('',*,*,#55807,.F.);
#83826=ORIENTED_EDGE('',*,*,#57702,.T.);
#83827=ORIENTED_EDGE('',*,*,#55808,.F.);
#83828=ORIENTED_EDGE('',*,*,#57703,.T.);
#83829=ORIENTED_EDGE('',*,*,#53334,.F.);
#83830=ORIENTED_EDGE('',*,*,#53330,.T.);
#83831=ORIENTED_EDGE('',*,*,#57704,.F.);
#83832=ORIENTED_EDGE('',*,*,#55848,.F.);
#83833=ORIENTED_EDGE('',*,*,#57705,.F.);
#83834=ORIENTED_EDGE('',*,*,#53286,.F.);
#83835=ORIENTED_EDGE('',*,*,#57705,.T.);
#83836=ORIENTED_EDGE('',*,*,#55847,.F.);
#83837=ORIENTED_EDGE('',*,*,#57706,.F.);
#83838=ORIENTED_EDGE('',*,*,#53295,.F.);
#83839=ORIENTED_EDGE('',*,*,#53285,.T.);
#83840=ORIENTED_EDGE('',*,*,#53289,.F.);
#83841=ORIENTED_EDGE('',*,*,#57707,.F.);
#83842=ORIENTED_EDGE('',*,*,#55849,.F.);
#83843=ORIENTED_EDGE('',*,*,#57704,.T.);
#83844=ORIENTED_EDGE('',*,*,#57706,.T.);
#83845=ORIENTED_EDGE('',*,*,#55846,.F.);
#83846=ORIENTED_EDGE('',*,*,#57708,.F.);
#83847=ORIENTED_EDGE('',*,*,#53280,.F.);
#83848=ORIENTED_EDGE('',*,*,#57707,.T.);
#83849=ORIENTED_EDGE('',*,*,#53293,.F.);
#83850=ORIENTED_EDGE('',*,*,#57709,.F.);
#83851=ORIENTED_EDGE('',*,*,#55838,.F.);
#83852=ORIENTED_EDGE('',*,*,#57708,.T.);
#83853=ORIENTED_EDGE('',*,*,#55845,.F.);
#83854=ORIENTED_EDGE('',*,*,#57710,.F.);
#83855=ORIENTED_EDGE('',*,*,#53297,.F.);
#83856=ORIENTED_EDGE('',*,*,#57709,.T.);
#83857=ORIENTED_EDGE('',*,*,#52324,.F.);
#83858=ORIENTED_EDGE('',*,*,#57711,.F.);
#83859=ORIENTED_EDGE('',*,*,#55839,.F.);
#83860=ORIENTED_EDGE('',*,*,#57710,.T.);
#83861=ORIENTED_EDGE('',*,*,#55844,.F.);
#83862=ORIENTED_EDGE('',*,*,#57712,.F.);
#83863=ORIENTED_EDGE('',*,*,#53272,.T.);
#83864=ORIENTED_EDGE('',*,*,#53276,.F.);
#83865=ORIENTED_EDGE('',*,*,#57711,.T.);
#83866=ORIENTED_EDGE('',*,*,#52323,.F.);
#83867=ORIENTED_EDGE('',*,*,#57713,.F.);
#83868=ORIENTED_EDGE('',*,*,#56464,.F.);
#83869=ORIENTED_EDGE('',*,*,#57712,.T.);
#83870=ORIENTED_EDGE('',*,*,#55843,.F.);
#83871=ORIENTED_EDGE('',*,*,#57714,.F.);
#83872=ORIENTED_EDGE('',*,*,#53273,.F.);
#83873=ORIENTED_EDGE('',*,*,#57713,.T.);
#83874=ORIENTED_EDGE('',*,*,#52322,.F.);
#83875=ORIENTED_EDGE('',*,*,#57715,.F.);
#83876=ORIENTED_EDGE('',*,*,#55823,.F.);
#83877=ORIENTED_EDGE('',*,*,#57714,.T.);
#83878=ORIENTED_EDGE('',*,*,#55842,.F.);
#83879=ORIENTED_EDGE('',*,*,#57716,.F.);
#83880=ORIENTED_EDGE('',*,*,#53291,.F.);
#83881=ORIENTED_EDGE('',*,*,#57715,.T.);
#83882=ORIENTED_EDGE('',*,*,#52321,.F.);
#83883=ORIENTED_EDGE('',*,*,#57717,.F.);
#83884=ORIENTED_EDGE('',*,*,#56466,.F.);
#83885=ORIENTED_EDGE('',*,*,#57716,.T.);
#83886=ORIENTED_EDGE('',*,*,#55841,.F.);
#83887=ORIENTED_EDGE('',*,*,#57718,.F.);
#83888=ORIENTED_EDGE('',*,*,#52703,.F.);
#83889=ORIENTED_EDGE('',*,*,#57717,.T.);
#83890=ORIENTED_EDGE('',*,*,#52320,.F.);
#83891=ORIENTED_EDGE('',*,*,#57719,.F.);
#83892=ORIENTED_EDGE('',*,*,#55829,.F.);
#83893=ORIENTED_EDGE('',*,*,#57718,.T.);
#83894=ORIENTED_EDGE('',*,*,#56465,.F.);
#83895=ORIENTED_EDGE('',*,*,#57720,.F.);
#83896=ORIENTED_EDGE('',*,*,#52704,.F.);
#83897=ORIENTED_EDGE('',*,*,#57719,.T.);
#83898=ORIENTED_EDGE('',*,*,#53322,.F.);
#83899=ORIENTED_EDGE('',*,*,#57721,.F.);
#83900=ORIENTED_EDGE('',*,*,#55830,.F.);
#83901=ORIENTED_EDGE('',*,*,#57720,.T.);
#83902=ORIENTED_EDGE('',*,*,#55825,.F.);
#83903=ORIENTED_EDGE('',*,*,#57722,.F.);
#83904=ORIENTED_EDGE('',*,*,#52705,.F.);
#83905=ORIENTED_EDGE('',*,*,#53317,.F.);
#83906=ORIENTED_EDGE('',*,*,#53313,.T.);
#83907=ORIENTED_EDGE('',*,*,#57723,.F.);
#83908=ORIENTED_EDGE('',*,*,#55831,.F.);
#83909=ORIENTED_EDGE('',*,*,#57721,.T.);
#83910=ORIENTED_EDGE('',*,*,#57722,.T.);
#83911=ORIENTED_EDGE('',*,*,#56467,.F.);
#83912=ORIENTED_EDGE('',*,*,#57724,.F.);
#83913=ORIENTED_EDGE('',*,*,#52706,.F.);
#83914=ORIENTED_EDGE('',*,*,#57723,.T.);
#83915=ORIENTED_EDGE('',*,*,#53312,.F.);
#83916=ORIENTED_EDGE('',*,*,#57725,.F.);
#83917=ORIENTED_EDGE('',*,*,#55832,.F.);
#83918=ORIENTED_EDGE('',*,*,#57724,.T.);
#83919=ORIENTED_EDGE('',*,*,#55827,.F.);
#83920=ORIENTED_EDGE('',*,*,#57726,.F.);
#83921=ORIENTED_EDGE('',*,*,#52707,.F.);
#83922=ORIENTED_EDGE('',*,*,#57725,.T.);
#83923=ORIENTED_EDGE('',*,*,#53324,.F.);
#83924=ORIENTED_EDGE('',*,*,#57727,.F.);
#83925=ORIENTED_EDGE('',*,*,#55833,.F.);
#83926=ORIENTED_EDGE('',*,*,#57726,.T.);
#83927=ORIENTED_EDGE('',*,*,#55826,.F.);
#83928=ORIENTED_EDGE('',*,*,#57728,.F.);
#83929=ORIENTED_EDGE('',*,*,#53320,.F.);
#83930=ORIENTED_EDGE('',*,*,#57727,.T.);
#83931=ORIENTED_EDGE('',*,*,#53308,.F.);
#83932=ORIENTED_EDGE('',*,*,#57729,.F.);
#83933=ORIENTED_EDGE('',*,*,#55834,.F.);
#83934=ORIENTED_EDGE('',*,*,#57728,.T.);
#83935=ORIENTED_EDGE('',*,*,#55837,.F.);
#83936=ORIENTED_EDGE('',*,*,#57730,.F.);
#83937=ORIENTED_EDGE('',*,*,#53299,.F.);
#83938=ORIENTED_EDGE('',*,*,#57729,.T.);
#83939=ORIENTED_EDGE('',*,*,#53326,.F.);
#83940=ORIENTED_EDGE('',*,*,#57731,.F.);
#83941=ORIENTED_EDGE('',*,*,#55835,.F.);
#83942=ORIENTED_EDGE('',*,*,#57730,.T.);
#83943=ORIENTED_EDGE('',*,*,#55836,.F.);
#83944=ORIENTED_EDGE('',*,*,#57731,.T.);
#83945=ORIENTED_EDGE('',*,*,#53304,.F.);
#83946=ORIENTED_EDGE('',*,*,#53300,.T.);
#83947=ORIENTED_EDGE('',*,*,#57732,.F.);
#83948=ORIENTED_EDGE('',*,*,#55876,.F.);
#83949=ORIENTED_EDGE('',*,*,#57733,.F.);
#83950=ORIENTED_EDGE('',*,*,#53256,.F.);
#83951=ORIENTED_EDGE('',*,*,#57733,.T.);
#83952=ORIENTED_EDGE('',*,*,#55875,.F.);
#83953=ORIENTED_EDGE('',*,*,#57734,.F.);
#83954=ORIENTED_EDGE('',*,*,#53265,.F.);
#83955=ORIENTED_EDGE('',*,*,#53255,.T.);
#83956=ORIENTED_EDGE('',*,*,#53259,.F.);
#83957=ORIENTED_EDGE('',*,*,#57735,.F.);
#83958=ORIENTED_EDGE('',*,*,#55877,.F.);
#83959=ORIENTED_EDGE('',*,*,#57732,.T.);
#83960=ORIENTED_EDGE('',*,*,#57734,.T.);
#83961=ORIENTED_EDGE('',*,*,#55874,.F.);
#83962=ORIENTED_EDGE('',*,*,#57736,.F.);
#83963=ORIENTED_EDGE('',*,*,#53250,.F.);
#83964=ORIENTED_EDGE('',*,*,#57735,.T.);
#83965=ORIENTED_EDGE('',*,*,#53263,.F.);
#83966=ORIENTED_EDGE('',*,*,#57737,.F.);
#83967=ORIENTED_EDGE('',*,*,#55866,.F.);
#83968=ORIENTED_EDGE('',*,*,#57736,.T.);
#83969=ORIENTED_EDGE('',*,*,#55873,.F.);
#83970=ORIENTED_EDGE('',*,*,#57738,.F.);
#83971=ORIENTED_EDGE('',*,*,#53267,.F.);
#83972=ORIENTED_EDGE('',*,*,#57737,.T.);
#83973=ORIENTED_EDGE('',*,*,#52330,.F.);
#83974=ORIENTED_EDGE('',*,*,#57739,.F.);
#83975=ORIENTED_EDGE('',*,*,#55867,.F.);
#83976=ORIENTED_EDGE('',*,*,#57738,.T.);
#83977=ORIENTED_EDGE('',*,*,#55872,.F.);
#83978=ORIENTED_EDGE('',*,*,#57740,.F.);
#83979=ORIENTED_EDGE('',*,*,#53242,.T.);
#83980=ORIENTED_EDGE('',*,*,#53246,.F.);
#83981=ORIENTED_EDGE('',*,*,#57739,.T.);
#83982=ORIENTED_EDGE('',*,*,#52329,.F.);
#83983=ORIENTED_EDGE('',*,*,#57741,.F.);
#83984=ORIENTED_EDGE('',*,*,#56468,.F.);
#83985=ORIENTED_EDGE('',*,*,#57740,.T.);
#83986=ORIENTED_EDGE('',*,*,#55871,.F.);
#83987=ORIENTED_EDGE('',*,*,#57742,.F.);
#83988=ORIENTED_EDGE('',*,*,#53243,.F.);
#83989=ORIENTED_EDGE('',*,*,#57741,.T.);
#83990=ORIENTED_EDGE('',*,*,#52328,.F.);
#83991=ORIENTED_EDGE('',*,*,#57743,.F.);
#83992=ORIENTED_EDGE('',*,*,#55851,.F.);
#83993=ORIENTED_EDGE('',*,*,#57742,.T.);
#83994=ORIENTED_EDGE('',*,*,#55870,.F.);
#83995=ORIENTED_EDGE('',*,*,#57744,.F.);
#83996=ORIENTED_EDGE('',*,*,#53261,.F.);
#83997=ORIENTED_EDGE('',*,*,#57743,.T.);
#83998=ORIENTED_EDGE('',*,*,#52327,.F.);
#83999=ORIENTED_EDGE('',*,*,#57745,.F.);
#84000=ORIENTED_EDGE('',*,*,#56470,.F.);
#84001=ORIENTED_EDGE('',*,*,#57744,.T.);
#84002=ORIENTED_EDGE('',*,*,#55869,.F.);
#84003=ORIENTED_EDGE('',*,*,#57746,.F.);
#84004=ORIENTED_EDGE('',*,*,#52697,.F.);
#84005=ORIENTED_EDGE('',*,*,#57745,.T.);
#84006=ORIENTED_EDGE('',*,*,#52326,.F.);
#84007=ORIENTED_EDGE('',*,*,#57747,.F.);
#84008=ORIENTED_EDGE('',*,*,#55857,.F.);
#84009=ORIENTED_EDGE('',*,*,#57746,.T.);
#84010=ORIENTED_EDGE('',*,*,#56469,.F.);
#84011=ORIENTED_EDGE('',*,*,#57748,.F.);
#84012=ORIENTED_EDGE('',*,*,#52698,.F.);
#84013=ORIENTED_EDGE('',*,*,#57747,.T.);
#84014=ORIENTED_EDGE('',*,*,#53292,.F.);
#84015=ORIENTED_EDGE('',*,*,#57749,.F.);
#84016=ORIENTED_EDGE('',*,*,#55858,.F.);
#84017=ORIENTED_EDGE('',*,*,#57748,.T.);
#84018=ORIENTED_EDGE('',*,*,#55853,.F.);
#84019=ORIENTED_EDGE('',*,*,#57750,.F.);
#84020=ORIENTED_EDGE('',*,*,#52699,.F.);
#84021=ORIENTED_EDGE('',*,*,#53287,.F.);
#84022=ORIENTED_EDGE('',*,*,#53283,.T.);
#84023=ORIENTED_EDGE('',*,*,#57751,.F.);
#84024=ORIENTED_EDGE('',*,*,#55859,.F.);
#84025=ORIENTED_EDGE('',*,*,#57749,.T.);
#84026=ORIENTED_EDGE('',*,*,#57750,.T.);
#84027=ORIENTED_EDGE('',*,*,#56471,.F.);
#84028=ORIENTED_EDGE('',*,*,#57752,.F.);
#84029=ORIENTED_EDGE('',*,*,#52700,.F.);
#84030=ORIENTED_EDGE('',*,*,#57751,.T.);
#84031=ORIENTED_EDGE('',*,*,#53282,.F.);
#84032=ORIENTED_EDGE('',*,*,#57753,.F.);
#84033=ORIENTED_EDGE('',*,*,#55860,.F.);
#84034=ORIENTED_EDGE('',*,*,#57752,.T.);
#84035=ORIENTED_EDGE('',*,*,#55855,.F.);
#84036=ORIENTED_EDGE('',*,*,#57754,.F.);
#84037=ORIENTED_EDGE('',*,*,#52701,.F.);
#84038=ORIENTED_EDGE('',*,*,#57753,.T.);
#84039=ORIENTED_EDGE('',*,*,#53294,.F.);
#84040=ORIENTED_EDGE('',*,*,#57755,.F.);
#84041=ORIENTED_EDGE('',*,*,#55861,.F.);
#84042=ORIENTED_EDGE('',*,*,#57754,.T.);
#84043=ORIENTED_EDGE('',*,*,#55854,.F.);
#84044=ORIENTED_EDGE('',*,*,#57756,.F.);
#84045=ORIENTED_EDGE('',*,*,#53290,.F.);
#84046=ORIENTED_EDGE('',*,*,#57755,.T.);
#84047=ORIENTED_EDGE('',*,*,#53278,.F.);
#84048=ORIENTED_EDGE('',*,*,#57757,.F.);
#84049=ORIENTED_EDGE('',*,*,#55862,.F.);
#84050=ORIENTED_EDGE('',*,*,#57756,.T.);
#84051=ORIENTED_EDGE('',*,*,#55865,.F.);
#84052=ORIENTED_EDGE('',*,*,#57758,.F.);
#84053=ORIENTED_EDGE('',*,*,#53269,.F.);
#84054=ORIENTED_EDGE('',*,*,#57757,.T.);
#84055=ORIENTED_EDGE('',*,*,#53296,.F.);
#84056=ORIENTED_EDGE('',*,*,#57759,.F.);
#84057=ORIENTED_EDGE('',*,*,#55863,.F.);
#84058=ORIENTED_EDGE('',*,*,#57758,.T.);
#84059=ORIENTED_EDGE('',*,*,#55864,.F.);
#84060=ORIENTED_EDGE('',*,*,#57759,.T.);
#84061=ORIENTED_EDGE('',*,*,#53274,.F.);
#84062=ORIENTED_EDGE('',*,*,#53270,.T.);
#84063=ORIENTED_EDGE('',*,*,#57760,.F.);
#84064=ORIENTED_EDGE('',*,*,#55902,.F.);
#84065=ORIENTED_EDGE('',*,*,#57761,.F.);
#84066=ORIENTED_EDGE('',*,*,#53226,.F.);
#84067=ORIENTED_EDGE('',*,*,#57761,.T.);
#84068=ORIENTED_EDGE('',*,*,#55901,.F.);
#84069=ORIENTED_EDGE('',*,*,#57762,.F.);
#84070=ORIENTED_EDGE('',*,*,#53235,.F.);
#84071=ORIENTED_EDGE('',*,*,#53225,.T.);
#84072=ORIENTED_EDGE('',*,*,#53229,.F.);
#84073=ORIENTED_EDGE('',*,*,#57763,.F.);
#84074=ORIENTED_EDGE('',*,*,#55903,.F.);
#84075=ORIENTED_EDGE('',*,*,#57760,.T.);
#84076=ORIENTED_EDGE('',*,*,#57762,.T.);
#84077=ORIENTED_EDGE('',*,*,#55900,.F.);
#84078=ORIENTED_EDGE('',*,*,#57764,.F.);
#84079=ORIENTED_EDGE('',*,*,#53220,.F.);
#84080=ORIENTED_EDGE('',*,*,#57763,.T.);
#84081=ORIENTED_EDGE('',*,*,#53233,.F.);
#84082=ORIENTED_EDGE('',*,*,#57765,.F.);
#84083=ORIENTED_EDGE('',*,*,#55892,.F.);
#84084=ORIENTED_EDGE('',*,*,#57764,.T.);
#84085=ORIENTED_EDGE('',*,*,#55899,.F.);
#84086=ORIENTED_EDGE('',*,*,#57766,.F.);
#84087=ORIENTED_EDGE('',*,*,#53237,.F.);
#84088=ORIENTED_EDGE('',*,*,#57765,.T.);
#84089=ORIENTED_EDGE('',*,*,#52335,.F.);
#84090=ORIENTED_EDGE('',*,*,#57767,.F.);
#84091=ORIENTED_EDGE('',*,*,#55893,.F.);
#84092=ORIENTED_EDGE('',*,*,#57766,.T.);
#84093=ORIENTED_EDGE('',*,*,#55898,.F.);
#84094=ORIENTED_EDGE('',*,*,#57768,.F.);
#84095=ORIENTED_EDGE('',*,*,#53212,.T.);
#84096=ORIENTED_EDGE('',*,*,#53216,.F.);
#84097=ORIENTED_EDGE('',*,*,#57767,.T.);
#84098=ORIENTED_EDGE('',*,*,#52334,.F.);
#84099=ORIENTED_EDGE('',*,*,#52036,.F.);
#84100=ORIENTED_EDGE('',*,*,#56472,.F.);
#84101=ORIENTED_EDGE('',*,*,#57768,.T.);
#84102=ORIENTED_EDGE('',*,*,#55897,.F.);
#84103=ORIENTED_EDGE('',*,*,#57769,.F.);
#84104=ORIENTED_EDGE('',*,*,#53213,.F.);
#84105=ORIENTED_EDGE('',*,*,#57769,.T.);
#84106=ORIENTED_EDGE('',*,*,#55896,.F.);
#84107=ORIENTED_EDGE('',*,*,#57770,.F.);
#84108=ORIENTED_EDGE('',*,*,#53231,.F.);
#84109=ORIENTED_EDGE('',*,*,#52034,.T.);
#84110=ORIENTED_EDGE('',*,*,#52333,.F.);
#84111=ORIENTED_EDGE('',*,*,#57771,.F.);
#84112=ORIENTED_EDGE('',*,*,#56474,.F.);
#84113=ORIENTED_EDGE('',*,*,#57770,.T.);
#84114=ORIENTED_EDGE('',*,*,#55895,.F.);
#84115=ORIENTED_EDGE('',*,*,#57772,.F.);
#84116=ORIENTED_EDGE('',*,*,#52692,.F.);
#84117=ORIENTED_EDGE('',*,*,#57771,.T.);
#84118=ORIENTED_EDGE('',*,*,#52332,.F.);
#84119=ORIENTED_EDGE('',*,*,#57773,.F.);
#84120=ORIENTED_EDGE('',*,*,#55883,.F.);
#84121=ORIENTED_EDGE('',*,*,#57772,.T.);
#84122=ORIENTED_EDGE('',*,*,#56473,.F.);
#84123=ORIENTED_EDGE('',*,*,#52032,.F.);
#84124=ORIENTED_EDGE('',*,*,#52693,.F.);
#84125=ORIENTED_EDGE('',*,*,#57773,.T.);
#84126=ORIENTED_EDGE('',*,*,#53262,.F.);
#84127=ORIENTED_EDGE('',*,*,#57774,.F.);
#84128=ORIENTED_EDGE('',*,*,#55884,.F.);
#84129=ORIENTED_EDGE('',*,*,#53257,.F.);
#84130=ORIENTED_EDGE('',*,*,#53253,.T.);
#84131=ORIENTED_EDGE('',*,*,#57775,.F.);
#84132=ORIENTED_EDGE('',*,*,#55885,.F.);
#84133=ORIENTED_EDGE('',*,*,#57774,.T.);
#84134=ORIENTED_EDGE('',*,*,#52030,.T.);
#84135=ORIENTED_EDGE('',*,*,#56475,.F.);
#84136=ORIENTED_EDGE('',*,*,#57776,.F.);
#84137=ORIENTED_EDGE('',*,*,#52694,.F.);
#84138=ORIENTED_EDGE('',*,*,#57775,.T.);
#84139=ORIENTED_EDGE('',*,*,#53252,.F.);
#84140=ORIENTED_EDGE('',*,*,#57777,.F.);
#84141=ORIENTED_EDGE('',*,*,#55886,.F.);
#84142=ORIENTED_EDGE('',*,*,#57776,.T.);
#84143=ORIENTED_EDGE('',*,*,#55881,.F.);
#84144=ORIENTED_EDGE('',*,*,#57778,.F.);
#84145=ORIENTED_EDGE('',*,*,#52695,.F.);
#84146=ORIENTED_EDGE('',*,*,#57777,.T.);
#84147=ORIENTED_EDGE('',*,*,#53264,.F.);
#84148=ORIENTED_EDGE('',*,*,#57779,.F.);
#84149=ORIENTED_EDGE('',*,*,#55887,.F.);
#84150=ORIENTED_EDGE('',*,*,#57778,.T.);
#84151=ORIENTED_EDGE('',*,*,#55880,.F.);
#84152=ORIENTED_EDGE('',*,*,#57780,.F.);
#84153=ORIENTED_EDGE('',*,*,#53260,.F.);
#84154=ORIENTED_EDGE('',*,*,#57779,.T.);
#84155=ORIENTED_EDGE('',*,*,#53248,.F.);
#84156=ORIENTED_EDGE('',*,*,#57781,.F.);
#84157=ORIENTED_EDGE('',*,*,#55888,.F.);
#84158=ORIENTED_EDGE('',*,*,#57780,.T.);
#84159=ORIENTED_EDGE('',*,*,#55891,.F.);
#84160=ORIENTED_EDGE('',*,*,#57782,.F.);
#84161=ORIENTED_EDGE('',*,*,#53239,.F.);
#84162=ORIENTED_EDGE('',*,*,#57781,.T.);
#84163=ORIENTED_EDGE('',*,*,#53266,.F.);
#84164=ORIENTED_EDGE('',*,*,#57783,.F.);
#84165=ORIENTED_EDGE('',*,*,#55889,.F.);
#84166=ORIENTED_EDGE('',*,*,#57782,.T.);
#84167=ORIENTED_EDGE('',*,*,#55890,.F.);
#84168=ORIENTED_EDGE('',*,*,#57783,.T.);
#84169=ORIENTED_EDGE('',*,*,#53244,.F.);
#84170=ORIENTED_EDGE('',*,*,#53240,.T.);
#84171=ORIENTED_EDGE('',*,*,#57784,.F.);
#84172=ORIENTED_EDGE('',*,*,#55930,.F.);
#84173=ORIENTED_EDGE('',*,*,#57785,.F.);
#84174=ORIENTED_EDGE('',*,*,#53196,.F.);
#84175=ORIENTED_EDGE('',*,*,#57785,.T.);
#84176=ORIENTED_EDGE('',*,*,#55929,.F.);
#84177=ORIENTED_EDGE('',*,*,#57786,.F.);
#84178=ORIENTED_EDGE('',*,*,#53205,.F.);
#84179=ORIENTED_EDGE('',*,*,#53195,.T.);
#84180=ORIENTED_EDGE('',*,*,#53199,.F.);
#84181=ORIENTED_EDGE('',*,*,#57787,.F.);
#84182=ORIENTED_EDGE('',*,*,#55931,.F.);
#84183=ORIENTED_EDGE('',*,*,#57784,.T.);
#84184=ORIENTED_EDGE('',*,*,#57786,.T.);
#84185=ORIENTED_EDGE('',*,*,#55928,.F.);
#84186=ORIENTED_EDGE('',*,*,#57788,.F.);
#84187=ORIENTED_EDGE('',*,*,#53190,.F.);
#84188=ORIENTED_EDGE('',*,*,#57787,.T.);
#84189=ORIENTED_EDGE('',*,*,#53203,.F.);
#84190=ORIENTED_EDGE('',*,*,#57789,.F.);
#84191=ORIENTED_EDGE('',*,*,#55920,.F.);
#84192=ORIENTED_EDGE('',*,*,#57788,.T.);
#84193=ORIENTED_EDGE('',*,*,#55927,.F.);
#84194=ORIENTED_EDGE('',*,*,#57790,.F.);
#84195=ORIENTED_EDGE('',*,*,#53207,.F.);
#84196=ORIENTED_EDGE('',*,*,#57789,.T.);
#84197=ORIENTED_EDGE('',*,*,#52341,.F.);
#84198=ORIENTED_EDGE('',*,*,#57791,.F.);
#84199=ORIENTED_EDGE('',*,*,#55921,.F.);
#84200=ORIENTED_EDGE('',*,*,#57790,.T.);
#84201=ORIENTED_EDGE('',*,*,#55926,.F.);
#84202=ORIENTED_EDGE('',*,*,#57792,.F.);
#84203=ORIENTED_EDGE('',*,*,#53182,.T.);
#84204=ORIENTED_EDGE('',*,*,#53186,.F.);
#84205=ORIENTED_EDGE('',*,*,#57791,.T.);
#84206=ORIENTED_EDGE('',*,*,#52340,.F.);
#84207=ORIENTED_EDGE('',*,*,#57793,.F.);
#84208=ORIENTED_EDGE('',*,*,#56476,.F.);
#84209=ORIENTED_EDGE('',*,*,#57792,.T.);
#84210=ORIENTED_EDGE('',*,*,#55925,.F.);
#84211=ORIENTED_EDGE('',*,*,#57794,.F.);
#84212=ORIENTED_EDGE('',*,*,#53183,.F.);
#84213=ORIENTED_EDGE('',*,*,#57793,.T.);
#84214=ORIENTED_EDGE('',*,*,#52339,.F.);
#84215=ORIENTED_EDGE('',*,*,#57795,.F.);
#84216=ORIENTED_EDGE('',*,*,#55905,.F.);
#84217=ORIENTED_EDGE('',*,*,#57794,.T.);
#84218=ORIENTED_EDGE('',*,*,#55924,.F.);
#84219=ORIENTED_EDGE('',*,*,#57796,.F.);
#84220=ORIENTED_EDGE('',*,*,#53201,.F.);
#84221=ORIENTED_EDGE('',*,*,#57795,.T.);
#84222=ORIENTED_EDGE('',*,*,#52338,.F.);
#84223=ORIENTED_EDGE('',*,*,#57797,.F.);
#84224=ORIENTED_EDGE('',*,*,#56478,.F.);
#84225=ORIENTED_EDGE('',*,*,#57796,.T.);
#84226=ORIENTED_EDGE('',*,*,#55923,.F.);
#84227=ORIENTED_EDGE('',*,*,#57798,.F.);
#84228=ORIENTED_EDGE('',*,*,#52686,.F.);
#84229=ORIENTED_EDGE('',*,*,#57797,.T.);
#84230=ORIENTED_EDGE('',*,*,#52337,.F.);
#84231=ORIENTED_EDGE('',*,*,#57799,.F.);
#84232=ORIENTED_EDGE('',*,*,#55911,.F.);
#84233=ORIENTED_EDGE('',*,*,#57798,.T.);
#84234=ORIENTED_EDGE('',*,*,#56477,.F.);
#84235=ORIENTED_EDGE('',*,*,#57800,.F.);
#84236=ORIENTED_EDGE('',*,*,#52687,.F.);
#84237=ORIENTED_EDGE('',*,*,#57799,.T.);
#84238=ORIENTED_EDGE('',*,*,#53232,.F.);
#84239=ORIENTED_EDGE('',*,*,#57801,.F.);
#84240=ORIENTED_EDGE('',*,*,#55912,.F.);
#84241=ORIENTED_EDGE('',*,*,#57800,.T.);
#84242=ORIENTED_EDGE('',*,*,#55907,.F.);
#84243=ORIENTED_EDGE('',*,*,#57802,.F.);
#84244=ORIENTED_EDGE('',*,*,#52688,.F.);
#84245=ORIENTED_EDGE('',*,*,#53227,.F.);
#84246=ORIENTED_EDGE('',*,*,#53223,.T.);
#84247=ORIENTED_EDGE('',*,*,#57803,.F.);
#84248=ORIENTED_EDGE('',*,*,#55913,.F.);
#84249=ORIENTED_EDGE('',*,*,#57801,.T.);
#84250=ORIENTED_EDGE('',*,*,#57802,.T.);
#84251=ORIENTED_EDGE('',*,*,#56479,.F.);
#84252=ORIENTED_EDGE('',*,*,#57804,.F.);
#84253=ORIENTED_EDGE('',*,*,#52689,.F.);
#84254=ORIENTED_EDGE('',*,*,#57803,.T.);
#84255=ORIENTED_EDGE('',*,*,#53222,.F.);
#84256=ORIENTED_EDGE('',*,*,#57805,.F.);
#84257=ORIENTED_EDGE('',*,*,#55914,.F.);
#84258=ORIENTED_EDGE('',*,*,#57804,.T.);
#84259=ORIENTED_EDGE('',*,*,#55909,.F.);
#84260=ORIENTED_EDGE('',*,*,#57806,.F.);
#84261=ORIENTED_EDGE('',*,*,#52690,.F.);
#84262=ORIENTED_EDGE('',*,*,#57805,.T.);
#84263=ORIENTED_EDGE('',*,*,#53234,.F.);
#84264=ORIENTED_EDGE('',*,*,#57807,.F.);
#84265=ORIENTED_EDGE('',*,*,#55915,.F.);
#84266=ORIENTED_EDGE('',*,*,#57806,.T.);
#84267=ORIENTED_EDGE('',*,*,#55908,.F.);
#84268=ORIENTED_EDGE('',*,*,#57808,.F.);
#84269=ORIENTED_EDGE('',*,*,#53230,.F.);
#84270=ORIENTED_EDGE('',*,*,#57807,.T.);
#84271=ORIENTED_EDGE('',*,*,#53218,.F.);
#84272=ORIENTED_EDGE('',*,*,#57809,.F.);
#84273=ORIENTED_EDGE('',*,*,#55916,.F.);
#84274=ORIENTED_EDGE('',*,*,#57808,.T.);
#84275=ORIENTED_EDGE('',*,*,#55919,.F.);
#84276=ORIENTED_EDGE('',*,*,#57810,.F.);
#84277=ORIENTED_EDGE('',*,*,#53209,.F.);
#84278=ORIENTED_EDGE('',*,*,#57809,.T.);
#84279=ORIENTED_EDGE('',*,*,#53236,.F.);
#84280=ORIENTED_EDGE('',*,*,#57811,.F.);
#84281=ORIENTED_EDGE('',*,*,#55917,.F.);
#84282=ORIENTED_EDGE('',*,*,#57810,.T.);
#84283=ORIENTED_EDGE('',*,*,#55918,.F.);
#84284=ORIENTED_EDGE('',*,*,#57811,.T.);
#84285=ORIENTED_EDGE('',*,*,#53214,.F.);
#84286=ORIENTED_EDGE('',*,*,#53210,.T.);
#84287=ORIENTED_EDGE('',*,*,#57812,.F.);
#84288=ORIENTED_EDGE('',*,*,#55958,.F.);
#84289=ORIENTED_EDGE('',*,*,#57813,.F.);
#84290=ORIENTED_EDGE('',*,*,#53166,.F.);
#84291=ORIENTED_EDGE('',*,*,#57813,.T.);
#84292=ORIENTED_EDGE('',*,*,#55957,.F.);
#84293=ORIENTED_EDGE('',*,*,#57814,.F.);
#84294=ORIENTED_EDGE('',*,*,#53175,.F.);
#84295=ORIENTED_EDGE('',*,*,#53165,.T.);
#84296=ORIENTED_EDGE('',*,*,#53169,.F.);
#84297=ORIENTED_EDGE('',*,*,#57815,.F.);
#84298=ORIENTED_EDGE('',*,*,#55959,.F.);
#84299=ORIENTED_EDGE('',*,*,#57812,.T.);
#84300=ORIENTED_EDGE('',*,*,#57814,.T.);
#84301=ORIENTED_EDGE('',*,*,#55956,.F.);
#84302=ORIENTED_EDGE('',*,*,#57816,.F.);
#84303=ORIENTED_EDGE('',*,*,#53160,.F.);
#84304=ORIENTED_EDGE('',*,*,#57815,.T.);
#84305=ORIENTED_EDGE('',*,*,#53173,.F.);
#84306=ORIENTED_EDGE('',*,*,#57817,.F.);
#84307=ORIENTED_EDGE('',*,*,#55948,.F.);
#84308=ORIENTED_EDGE('',*,*,#57816,.T.);
#84309=ORIENTED_EDGE('',*,*,#55955,.F.);
#84310=ORIENTED_EDGE('',*,*,#57818,.F.);
#84311=ORIENTED_EDGE('',*,*,#53177,.F.);
#84312=ORIENTED_EDGE('',*,*,#57817,.T.);
#84313=ORIENTED_EDGE('',*,*,#52347,.F.);
#84314=ORIENTED_EDGE('',*,*,#57819,.F.);
#84315=ORIENTED_EDGE('',*,*,#55949,.F.);
#84316=ORIENTED_EDGE('',*,*,#57818,.T.);
#84317=ORIENTED_EDGE('',*,*,#55954,.F.);
#84318=ORIENTED_EDGE('',*,*,#57820,.F.);
#84319=ORIENTED_EDGE('',*,*,#53152,.T.);
#84320=ORIENTED_EDGE('',*,*,#53156,.F.);
#84321=ORIENTED_EDGE('',*,*,#57819,.T.);
#84322=ORIENTED_EDGE('',*,*,#52346,.F.);
#84323=ORIENTED_EDGE('',*,*,#57821,.F.);
#84324=ORIENTED_EDGE('',*,*,#56480,.F.);
#84325=ORIENTED_EDGE('',*,*,#57820,.T.);
#84326=ORIENTED_EDGE('',*,*,#55953,.F.);
#84327=ORIENTED_EDGE('',*,*,#57822,.F.);
#84328=ORIENTED_EDGE('',*,*,#53153,.F.);
#84329=ORIENTED_EDGE('',*,*,#57821,.T.);
#84330=ORIENTED_EDGE('',*,*,#52345,.F.);
#84331=ORIENTED_EDGE('',*,*,#57823,.F.);
#84332=ORIENTED_EDGE('',*,*,#55933,.F.);
#84333=ORIENTED_EDGE('',*,*,#57822,.T.);
#84334=ORIENTED_EDGE('',*,*,#55952,.F.);
#84335=ORIENTED_EDGE('',*,*,#57824,.F.);
#84336=ORIENTED_EDGE('',*,*,#53171,.F.);
#84337=ORIENTED_EDGE('',*,*,#57823,.T.);
#84338=ORIENTED_EDGE('',*,*,#52344,.F.);
#84339=ORIENTED_EDGE('',*,*,#57825,.F.);
#84340=ORIENTED_EDGE('',*,*,#56482,.F.);
#84341=ORIENTED_EDGE('',*,*,#57824,.T.);
#84342=ORIENTED_EDGE('',*,*,#55951,.F.);
#84343=ORIENTED_EDGE('',*,*,#57826,.F.);
#84344=ORIENTED_EDGE('',*,*,#52680,.F.);
#84345=ORIENTED_EDGE('',*,*,#57825,.T.);
#84346=ORIENTED_EDGE('',*,*,#52343,.F.);
#84347=ORIENTED_EDGE('',*,*,#57827,.F.);
#84348=ORIENTED_EDGE('',*,*,#55939,.F.);
#84349=ORIENTED_EDGE('',*,*,#57826,.T.);
#84350=ORIENTED_EDGE('',*,*,#56481,.F.);
#84351=ORIENTED_EDGE('',*,*,#57828,.F.);
#84352=ORIENTED_EDGE('',*,*,#52681,.F.);
#84353=ORIENTED_EDGE('',*,*,#57827,.T.);
#84354=ORIENTED_EDGE('',*,*,#53202,.F.);
#84355=ORIENTED_EDGE('',*,*,#57829,.F.);
#84356=ORIENTED_EDGE('',*,*,#55940,.F.);
#84357=ORIENTED_EDGE('',*,*,#57828,.T.);
#84358=ORIENTED_EDGE('',*,*,#55935,.F.);
#84359=ORIENTED_EDGE('',*,*,#57830,.F.);
#84360=ORIENTED_EDGE('',*,*,#52682,.F.);
#84361=ORIENTED_EDGE('',*,*,#53197,.F.);
#84362=ORIENTED_EDGE('',*,*,#53193,.T.);
#84363=ORIENTED_EDGE('',*,*,#57831,.F.);
#84364=ORIENTED_EDGE('',*,*,#55941,.F.);
#84365=ORIENTED_EDGE('',*,*,#57829,.T.);
#84366=ORIENTED_EDGE('',*,*,#57830,.T.);
#84367=ORIENTED_EDGE('',*,*,#56483,.F.);
#84368=ORIENTED_EDGE('',*,*,#57832,.F.);
#84369=ORIENTED_EDGE('',*,*,#52683,.F.);
#84370=ORIENTED_EDGE('',*,*,#57831,.T.);
#84371=ORIENTED_EDGE('',*,*,#53192,.F.);
#84372=ORIENTED_EDGE('',*,*,#57833,.F.);
#84373=ORIENTED_EDGE('',*,*,#55942,.F.);
#84374=ORIENTED_EDGE('',*,*,#57832,.T.);
#84375=ORIENTED_EDGE('',*,*,#55937,.F.);
#84376=ORIENTED_EDGE('',*,*,#57834,.F.);
#84377=ORIENTED_EDGE('',*,*,#52684,.F.);
#84378=ORIENTED_EDGE('',*,*,#57833,.T.);
#84379=ORIENTED_EDGE('',*,*,#53204,.F.);
#84380=ORIENTED_EDGE('',*,*,#57835,.F.);
#84381=ORIENTED_EDGE('',*,*,#55943,.F.);
#84382=ORIENTED_EDGE('',*,*,#57834,.T.);
#84383=ORIENTED_EDGE('',*,*,#55936,.F.);
#84384=ORIENTED_EDGE('',*,*,#57836,.F.);
#84385=ORIENTED_EDGE('',*,*,#53200,.F.);
#84386=ORIENTED_EDGE('',*,*,#57835,.T.);
#84387=ORIENTED_EDGE('',*,*,#53188,.F.);
#84388=ORIENTED_EDGE('',*,*,#57837,.F.);
#84389=ORIENTED_EDGE('',*,*,#55944,.F.);
#84390=ORIENTED_EDGE('',*,*,#57836,.T.);
#84391=ORIENTED_EDGE('',*,*,#55947,.F.);
#84392=ORIENTED_EDGE('',*,*,#57838,.F.);
#84393=ORIENTED_EDGE('',*,*,#53179,.F.);
#84394=ORIENTED_EDGE('',*,*,#57837,.T.);
#84395=ORIENTED_EDGE('',*,*,#53206,.F.);
#84396=ORIENTED_EDGE('',*,*,#57839,.F.);
#84397=ORIENTED_EDGE('',*,*,#55945,.F.);
#84398=ORIENTED_EDGE('',*,*,#57838,.T.);
#84399=ORIENTED_EDGE('',*,*,#55946,.F.);
#84400=ORIENTED_EDGE('',*,*,#57839,.T.);
#84401=ORIENTED_EDGE('',*,*,#53184,.F.);
#84402=ORIENTED_EDGE('',*,*,#53180,.T.);
#84403=ORIENTED_EDGE('',*,*,#57840,.F.);
#84404=ORIENTED_EDGE('',*,*,#55986,.F.);
#84405=ORIENTED_EDGE('',*,*,#57841,.F.);
#84406=ORIENTED_EDGE('',*,*,#53136,.F.);
#84407=ORIENTED_EDGE('',*,*,#57841,.T.);
#84408=ORIENTED_EDGE('',*,*,#55985,.F.);
#84409=ORIENTED_EDGE('',*,*,#57842,.F.);
#84410=ORIENTED_EDGE('',*,*,#53145,.F.);
#84411=ORIENTED_EDGE('',*,*,#53135,.T.);
#84412=ORIENTED_EDGE('',*,*,#53139,.F.);
#84413=ORIENTED_EDGE('',*,*,#57843,.F.);
#84414=ORIENTED_EDGE('',*,*,#55987,.F.);
#84415=ORIENTED_EDGE('',*,*,#57840,.T.);
#84416=ORIENTED_EDGE('',*,*,#57842,.T.);
#84417=ORIENTED_EDGE('',*,*,#55984,.F.);
#84418=ORIENTED_EDGE('',*,*,#57844,.F.);
#84419=ORIENTED_EDGE('',*,*,#53130,.F.);
#84420=ORIENTED_EDGE('',*,*,#57843,.T.);
#84421=ORIENTED_EDGE('',*,*,#53143,.F.);
#84422=ORIENTED_EDGE('',*,*,#57845,.F.);
#84423=ORIENTED_EDGE('',*,*,#55976,.F.);
#84424=ORIENTED_EDGE('',*,*,#57844,.T.);
#84425=ORIENTED_EDGE('',*,*,#55983,.F.);
#84426=ORIENTED_EDGE('',*,*,#57846,.F.);
#84427=ORIENTED_EDGE('',*,*,#53147,.F.);
#84428=ORIENTED_EDGE('',*,*,#57845,.T.);
#84429=ORIENTED_EDGE('',*,*,#52353,.F.);
#84430=ORIENTED_EDGE('',*,*,#57847,.F.);
#84431=ORIENTED_EDGE('',*,*,#55977,.F.);
#84432=ORIENTED_EDGE('',*,*,#57846,.T.);
#84433=ORIENTED_EDGE('',*,*,#55982,.F.);
#84434=ORIENTED_EDGE('',*,*,#57848,.F.);
#84435=ORIENTED_EDGE('',*,*,#53122,.T.);
#84436=ORIENTED_EDGE('',*,*,#53126,.F.);
#84437=ORIENTED_EDGE('',*,*,#57847,.T.);
#84438=ORIENTED_EDGE('',*,*,#52352,.F.);
#84439=ORIENTED_EDGE('',*,*,#57849,.F.);
#84440=ORIENTED_EDGE('',*,*,#56484,.F.);
#84441=ORIENTED_EDGE('',*,*,#57848,.T.);
#84442=ORIENTED_EDGE('',*,*,#55981,.F.);
#84443=ORIENTED_EDGE('',*,*,#57850,.F.);
#84444=ORIENTED_EDGE('',*,*,#53123,.F.);
#84445=ORIENTED_EDGE('',*,*,#57849,.T.);
#84446=ORIENTED_EDGE('',*,*,#52351,.F.);
#84447=ORIENTED_EDGE('',*,*,#57851,.F.);
#84448=ORIENTED_EDGE('',*,*,#55961,.F.);
#84449=ORIENTED_EDGE('',*,*,#57850,.T.);
#84450=ORIENTED_EDGE('',*,*,#55980,.F.);
#84451=ORIENTED_EDGE('',*,*,#57852,.F.);
#84452=ORIENTED_EDGE('',*,*,#53141,.F.);
#84453=ORIENTED_EDGE('',*,*,#57851,.T.);
#84454=ORIENTED_EDGE('',*,*,#52350,.F.);
#84455=ORIENTED_EDGE('',*,*,#57853,.F.);
#84456=ORIENTED_EDGE('',*,*,#56486,.F.);
#84457=ORIENTED_EDGE('',*,*,#57852,.T.);
#84458=ORIENTED_EDGE('',*,*,#55979,.F.);
#84459=ORIENTED_EDGE('',*,*,#57854,.F.);
#84460=ORIENTED_EDGE('',*,*,#52674,.F.);
#84461=ORIENTED_EDGE('',*,*,#57853,.T.);
#84462=ORIENTED_EDGE('',*,*,#52349,.F.);
#84463=ORIENTED_EDGE('',*,*,#57855,.F.);
#84464=ORIENTED_EDGE('',*,*,#55967,.F.);
#84465=ORIENTED_EDGE('',*,*,#57854,.T.);
#84466=ORIENTED_EDGE('',*,*,#56485,.F.);
#84467=ORIENTED_EDGE('',*,*,#57856,.F.);
#84468=ORIENTED_EDGE('',*,*,#52675,.F.);
#84469=ORIENTED_EDGE('',*,*,#57855,.T.);
#84470=ORIENTED_EDGE('',*,*,#53172,.F.);
#84471=ORIENTED_EDGE('',*,*,#57857,.F.);
#84472=ORIENTED_EDGE('',*,*,#55968,.F.);
#84473=ORIENTED_EDGE('',*,*,#57856,.T.);
#84474=ORIENTED_EDGE('',*,*,#55963,.F.);
#84475=ORIENTED_EDGE('',*,*,#57858,.F.);
#84476=ORIENTED_EDGE('',*,*,#52676,.F.);
#84477=ORIENTED_EDGE('',*,*,#53167,.F.);
#84478=ORIENTED_EDGE('',*,*,#53163,.T.);
#84479=ORIENTED_EDGE('',*,*,#57859,.F.);
#84480=ORIENTED_EDGE('',*,*,#55969,.F.);
#84481=ORIENTED_EDGE('',*,*,#57857,.T.);
#84482=ORIENTED_EDGE('',*,*,#57858,.T.);
#84483=ORIENTED_EDGE('',*,*,#56487,.F.);
#84484=ORIENTED_EDGE('',*,*,#57860,.F.);
#84485=ORIENTED_EDGE('',*,*,#52677,.F.);
#84486=ORIENTED_EDGE('',*,*,#57859,.T.);
#84487=ORIENTED_EDGE('',*,*,#53162,.F.);
#84488=ORIENTED_EDGE('',*,*,#57861,.F.);
#84489=ORIENTED_EDGE('',*,*,#55970,.F.);
#84490=ORIENTED_EDGE('',*,*,#57860,.T.);
#84491=ORIENTED_EDGE('',*,*,#55965,.F.);
#84492=ORIENTED_EDGE('',*,*,#57862,.F.);
#84493=ORIENTED_EDGE('',*,*,#52678,.F.);
#84494=ORIENTED_EDGE('',*,*,#57861,.T.);
#84495=ORIENTED_EDGE('',*,*,#53174,.F.);
#84496=ORIENTED_EDGE('',*,*,#57863,.F.);
#84497=ORIENTED_EDGE('',*,*,#55971,.F.);
#84498=ORIENTED_EDGE('',*,*,#57862,.T.);
#84499=ORIENTED_EDGE('',*,*,#55964,.F.);
#84500=ORIENTED_EDGE('',*,*,#57864,.F.);
#84501=ORIENTED_EDGE('',*,*,#53170,.F.);
#84502=ORIENTED_EDGE('',*,*,#57863,.T.);
#84503=ORIENTED_EDGE('',*,*,#53158,.F.);
#84504=ORIENTED_EDGE('',*,*,#57865,.F.);
#84505=ORIENTED_EDGE('',*,*,#55972,.F.);
#84506=ORIENTED_EDGE('',*,*,#57864,.T.);
#84507=ORIENTED_EDGE('',*,*,#55975,.F.);
#84508=ORIENTED_EDGE('',*,*,#57866,.F.);
#84509=ORIENTED_EDGE('',*,*,#53149,.F.);
#84510=ORIENTED_EDGE('',*,*,#57865,.T.);
#84511=ORIENTED_EDGE('',*,*,#53176,.F.);
#84512=ORIENTED_EDGE('',*,*,#57867,.F.);
#84513=ORIENTED_EDGE('',*,*,#55973,.F.);
#84514=ORIENTED_EDGE('',*,*,#57866,.T.);
#84515=ORIENTED_EDGE('',*,*,#55974,.F.);
#84516=ORIENTED_EDGE('',*,*,#57867,.T.);
#84517=ORIENTED_EDGE('',*,*,#53154,.F.);
#84518=ORIENTED_EDGE('',*,*,#53150,.T.);
#84519=ORIENTED_EDGE('',*,*,#57868,.F.);
#84520=ORIENTED_EDGE('',*,*,#56014,.F.);
#84521=ORIENTED_EDGE('',*,*,#57869,.F.);
#84522=ORIENTED_EDGE('',*,*,#53106,.F.);
#84523=ORIENTED_EDGE('',*,*,#57869,.T.);
#84524=ORIENTED_EDGE('',*,*,#56013,.F.);
#84525=ORIENTED_EDGE('',*,*,#57870,.F.);
#84526=ORIENTED_EDGE('',*,*,#53115,.F.);
#84527=ORIENTED_EDGE('',*,*,#53105,.T.);
#84528=ORIENTED_EDGE('',*,*,#53109,.F.);
#84529=ORIENTED_EDGE('',*,*,#57871,.F.);
#84530=ORIENTED_EDGE('',*,*,#56015,.F.);
#84531=ORIENTED_EDGE('',*,*,#57868,.T.);
#84532=ORIENTED_EDGE('',*,*,#57870,.T.);
#84533=ORIENTED_EDGE('',*,*,#56012,.F.);
#84534=ORIENTED_EDGE('',*,*,#57872,.F.);
#84535=ORIENTED_EDGE('',*,*,#53100,.F.);
#84536=ORIENTED_EDGE('',*,*,#57871,.T.);
#84537=ORIENTED_EDGE('',*,*,#53113,.F.);
#84538=ORIENTED_EDGE('',*,*,#57873,.F.);
#84539=ORIENTED_EDGE('',*,*,#56004,.F.);
#84540=ORIENTED_EDGE('',*,*,#57872,.T.);
#84541=ORIENTED_EDGE('',*,*,#56011,.F.);
#84542=ORIENTED_EDGE('',*,*,#57874,.F.);
#84543=ORIENTED_EDGE('',*,*,#53117,.F.);
#84544=ORIENTED_EDGE('',*,*,#57873,.T.);
#84545=ORIENTED_EDGE('',*,*,#52359,.F.);
#84546=ORIENTED_EDGE('',*,*,#57875,.F.);
#84547=ORIENTED_EDGE('',*,*,#56005,.F.);
#84548=ORIENTED_EDGE('',*,*,#57874,.T.);
#84549=ORIENTED_EDGE('',*,*,#56010,.F.);
#84550=ORIENTED_EDGE('',*,*,#57876,.F.);
#84551=ORIENTED_EDGE('',*,*,#53092,.T.);
#84552=ORIENTED_EDGE('',*,*,#53096,.F.);
#84553=ORIENTED_EDGE('',*,*,#57875,.T.);
#84554=ORIENTED_EDGE('',*,*,#52358,.F.);
#84555=ORIENTED_EDGE('',*,*,#57877,.F.);
#84556=ORIENTED_EDGE('',*,*,#56488,.F.);
#84557=ORIENTED_EDGE('',*,*,#57876,.T.);
#84558=ORIENTED_EDGE('',*,*,#56009,.F.);
#84559=ORIENTED_EDGE('',*,*,#57878,.F.);
#84560=ORIENTED_EDGE('',*,*,#53093,.F.);
#84561=ORIENTED_EDGE('',*,*,#57877,.T.);
#84562=ORIENTED_EDGE('',*,*,#52357,.F.);
#84563=ORIENTED_EDGE('',*,*,#57879,.F.);
#84564=ORIENTED_EDGE('',*,*,#55989,.F.);
#84565=ORIENTED_EDGE('',*,*,#57878,.T.);
#84566=ORIENTED_EDGE('',*,*,#56008,.F.);
#84567=ORIENTED_EDGE('',*,*,#57880,.F.);
#84568=ORIENTED_EDGE('',*,*,#53111,.F.);
#84569=ORIENTED_EDGE('',*,*,#57879,.T.);
#84570=ORIENTED_EDGE('',*,*,#52356,.F.);
#84571=ORIENTED_EDGE('',*,*,#57881,.F.);
#84572=ORIENTED_EDGE('',*,*,#56490,.F.);
#84573=ORIENTED_EDGE('',*,*,#57880,.T.);
#84574=ORIENTED_EDGE('',*,*,#56007,.F.);
#84575=ORIENTED_EDGE('',*,*,#57882,.F.);
#84576=ORIENTED_EDGE('',*,*,#52668,.F.);
#84577=ORIENTED_EDGE('',*,*,#57881,.T.);
#84578=ORIENTED_EDGE('',*,*,#52355,.F.);
#84579=ORIENTED_EDGE('',*,*,#57883,.F.);
#84580=ORIENTED_EDGE('',*,*,#55995,.F.);
#84581=ORIENTED_EDGE('',*,*,#57882,.T.);
#84582=ORIENTED_EDGE('',*,*,#56489,.F.);
#84583=ORIENTED_EDGE('',*,*,#57884,.F.);
#84584=ORIENTED_EDGE('',*,*,#52669,.F.);
#84585=ORIENTED_EDGE('',*,*,#57883,.T.);
#84586=ORIENTED_EDGE('',*,*,#53142,.F.);
#84587=ORIENTED_EDGE('',*,*,#57885,.F.);
#84588=ORIENTED_EDGE('',*,*,#55996,.F.);
#84589=ORIENTED_EDGE('',*,*,#57884,.T.);
#84590=ORIENTED_EDGE('',*,*,#55991,.F.);
#84591=ORIENTED_EDGE('',*,*,#57886,.F.);
#84592=ORIENTED_EDGE('',*,*,#52670,.F.);
#84593=ORIENTED_EDGE('',*,*,#53137,.F.);
#84594=ORIENTED_EDGE('',*,*,#53133,.T.);
#84595=ORIENTED_EDGE('',*,*,#57887,.F.);
#84596=ORIENTED_EDGE('',*,*,#55997,.F.);
#84597=ORIENTED_EDGE('',*,*,#57885,.T.);
#84598=ORIENTED_EDGE('',*,*,#57886,.T.);
#84599=ORIENTED_EDGE('',*,*,#56491,.F.);
#84600=ORIENTED_EDGE('',*,*,#57888,.F.);
#84601=ORIENTED_EDGE('',*,*,#52671,.F.);
#84602=ORIENTED_EDGE('',*,*,#57887,.T.);
#84603=ORIENTED_EDGE('',*,*,#53132,.F.);
#84604=ORIENTED_EDGE('',*,*,#57889,.F.);
#84605=ORIENTED_EDGE('',*,*,#55998,.F.);
#84606=ORIENTED_EDGE('',*,*,#57888,.T.);
#84607=ORIENTED_EDGE('',*,*,#55993,.F.);
#84608=ORIENTED_EDGE('',*,*,#57890,.F.);
#84609=ORIENTED_EDGE('',*,*,#52672,.F.);
#84610=ORIENTED_EDGE('',*,*,#57889,.T.);
#84611=ORIENTED_EDGE('',*,*,#53144,.F.);
#84612=ORIENTED_EDGE('',*,*,#57891,.F.);
#84613=ORIENTED_EDGE('',*,*,#55999,.F.);
#84614=ORIENTED_EDGE('',*,*,#57890,.T.);
#84615=ORIENTED_EDGE('',*,*,#55992,.F.);
#84616=ORIENTED_EDGE('',*,*,#57892,.F.);
#84617=ORIENTED_EDGE('',*,*,#53140,.F.);
#84618=ORIENTED_EDGE('',*,*,#57891,.T.);
#84619=ORIENTED_EDGE('',*,*,#53128,.F.);
#84620=ORIENTED_EDGE('',*,*,#57893,.F.);
#84621=ORIENTED_EDGE('',*,*,#56000,.F.);
#84622=ORIENTED_EDGE('',*,*,#57892,.T.);
#84623=ORIENTED_EDGE('',*,*,#56003,.F.);
#84624=ORIENTED_EDGE('',*,*,#57894,.F.);
#84625=ORIENTED_EDGE('',*,*,#53119,.F.);
#84626=ORIENTED_EDGE('',*,*,#57893,.T.);
#84627=ORIENTED_EDGE('',*,*,#53146,.F.);
#84628=ORIENTED_EDGE('',*,*,#57895,.F.);
#84629=ORIENTED_EDGE('',*,*,#56001,.F.);
#84630=ORIENTED_EDGE('',*,*,#57894,.T.);
#84631=ORIENTED_EDGE('',*,*,#56002,.F.);
#84632=ORIENTED_EDGE('',*,*,#57895,.T.);
#84633=ORIENTED_EDGE('',*,*,#53124,.F.);
#84634=ORIENTED_EDGE('',*,*,#53120,.T.);
#84635=ORIENTED_EDGE('',*,*,#57896,.F.);
#84636=ORIENTED_EDGE('',*,*,#56042,.F.);
#84637=ORIENTED_EDGE('',*,*,#57897,.F.);
#84638=ORIENTED_EDGE('',*,*,#53076,.F.);
#84639=ORIENTED_EDGE('',*,*,#57897,.T.);
#84640=ORIENTED_EDGE('',*,*,#56041,.F.);
#84641=ORIENTED_EDGE('',*,*,#57898,.F.);
#84642=ORIENTED_EDGE('',*,*,#53085,.F.);
#84643=ORIENTED_EDGE('',*,*,#53075,.T.);
#84644=ORIENTED_EDGE('',*,*,#53079,.F.);
#84645=ORIENTED_EDGE('',*,*,#57899,.F.);
#84646=ORIENTED_EDGE('',*,*,#56043,.F.);
#84647=ORIENTED_EDGE('',*,*,#57896,.T.);
#84648=ORIENTED_EDGE('',*,*,#57898,.T.);
#84649=ORIENTED_EDGE('',*,*,#56040,.F.);
#84650=ORIENTED_EDGE('',*,*,#57900,.F.);
#84651=ORIENTED_EDGE('',*,*,#53070,.F.);
#84652=ORIENTED_EDGE('',*,*,#57899,.T.);
#84653=ORIENTED_EDGE('',*,*,#53083,.F.);
#84654=ORIENTED_EDGE('',*,*,#57901,.F.);
#84655=ORIENTED_EDGE('',*,*,#56032,.F.);
#84656=ORIENTED_EDGE('',*,*,#57900,.T.);
#84657=ORIENTED_EDGE('',*,*,#56039,.F.);
#84658=ORIENTED_EDGE('',*,*,#57902,.F.);
#84659=ORIENTED_EDGE('',*,*,#53087,.F.);
#84660=ORIENTED_EDGE('',*,*,#57901,.T.);
#84661=ORIENTED_EDGE('',*,*,#52365,.F.);
#84662=ORIENTED_EDGE('',*,*,#57903,.F.);
#84663=ORIENTED_EDGE('',*,*,#56033,.F.);
#84664=ORIENTED_EDGE('',*,*,#57902,.T.);
#84665=ORIENTED_EDGE('',*,*,#56038,.F.);
#84666=ORIENTED_EDGE('',*,*,#57904,.F.);
#84667=ORIENTED_EDGE('',*,*,#53062,.T.);
#84668=ORIENTED_EDGE('',*,*,#53066,.F.);
#84669=ORIENTED_EDGE('',*,*,#57903,.T.);
#84670=ORIENTED_EDGE('',*,*,#52364,.F.);
#84671=ORIENTED_EDGE('',*,*,#57905,.F.);
#84672=ORIENTED_EDGE('',*,*,#56492,.F.);
#84673=ORIENTED_EDGE('',*,*,#57904,.T.);
#84674=ORIENTED_EDGE('',*,*,#56037,.F.);
#84675=ORIENTED_EDGE('',*,*,#57906,.F.);
#84676=ORIENTED_EDGE('',*,*,#53063,.F.);
#84677=ORIENTED_EDGE('',*,*,#57905,.T.);
#84678=ORIENTED_EDGE('',*,*,#52363,.F.);
#84679=ORIENTED_EDGE('',*,*,#57907,.F.);
#84680=ORIENTED_EDGE('',*,*,#56017,.F.);
#84681=ORIENTED_EDGE('',*,*,#57906,.T.);
#84682=ORIENTED_EDGE('',*,*,#56036,.F.);
#84683=ORIENTED_EDGE('',*,*,#57908,.F.);
#84684=ORIENTED_EDGE('',*,*,#53081,.F.);
#84685=ORIENTED_EDGE('',*,*,#57907,.T.);
#84686=ORIENTED_EDGE('',*,*,#52362,.F.);
#84687=ORIENTED_EDGE('',*,*,#57909,.F.);
#84688=ORIENTED_EDGE('',*,*,#56494,.F.);
#84689=ORIENTED_EDGE('',*,*,#57908,.T.);
#84690=ORIENTED_EDGE('',*,*,#56035,.F.);
#84691=ORIENTED_EDGE('',*,*,#57910,.F.);
#84692=ORIENTED_EDGE('',*,*,#52662,.F.);
#84693=ORIENTED_EDGE('',*,*,#57909,.T.);
#84694=ORIENTED_EDGE('',*,*,#52361,.F.);
#84695=ORIENTED_EDGE('',*,*,#57911,.F.);
#84696=ORIENTED_EDGE('',*,*,#56023,.F.);
#84697=ORIENTED_EDGE('',*,*,#57910,.T.);
#84698=ORIENTED_EDGE('',*,*,#56493,.F.);
#84699=ORIENTED_EDGE('',*,*,#57912,.F.);
#84700=ORIENTED_EDGE('',*,*,#52663,.F.);
#84701=ORIENTED_EDGE('',*,*,#57911,.T.);
#84702=ORIENTED_EDGE('',*,*,#53112,.F.);
#84703=ORIENTED_EDGE('',*,*,#57913,.F.);
#84704=ORIENTED_EDGE('',*,*,#56024,.F.);
#84705=ORIENTED_EDGE('',*,*,#57912,.T.);
#84706=ORIENTED_EDGE('',*,*,#56019,.F.);
#84707=ORIENTED_EDGE('',*,*,#57914,.F.);
#84708=ORIENTED_EDGE('',*,*,#52664,.F.);
#84709=ORIENTED_EDGE('',*,*,#53107,.F.);
#84710=ORIENTED_EDGE('',*,*,#53103,.T.);
#84711=ORIENTED_EDGE('',*,*,#57915,.F.);
#84712=ORIENTED_EDGE('',*,*,#56025,.F.);
#84713=ORIENTED_EDGE('',*,*,#57913,.T.);
#84714=ORIENTED_EDGE('',*,*,#57914,.T.);
#84715=ORIENTED_EDGE('',*,*,#56495,.F.);
#84716=ORIENTED_EDGE('',*,*,#57916,.F.);
#84717=ORIENTED_EDGE('',*,*,#52665,.F.);
#84718=ORIENTED_EDGE('',*,*,#57915,.T.);
#84719=ORIENTED_EDGE('',*,*,#53102,.F.);
#84720=ORIENTED_EDGE('',*,*,#57917,.F.);
#84721=ORIENTED_EDGE('',*,*,#56026,.F.);
#84722=ORIENTED_EDGE('',*,*,#57916,.T.);
#84723=ORIENTED_EDGE('',*,*,#56021,.F.);
#84724=ORIENTED_EDGE('',*,*,#57918,.F.);
#84725=ORIENTED_EDGE('',*,*,#52666,.F.);
#84726=ORIENTED_EDGE('',*,*,#57917,.T.);
#84727=ORIENTED_EDGE('',*,*,#53114,.F.);
#84728=ORIENTED_EDGE('',*,*,#57919,.F.);
#84729=ORIENTED_EDGE('',*,*,#56027,.F.);
#84730=ORIENTED_EDGE('',*,*,#57918,.T.);
#84731=ORIENTED_EDGE('',*,*,#56020,.F.);
#84732=ORIENTED_EDGE('',*,*,#57920,.F.);
#84733=ORIENTED_EDGE('',*,*,#53110,.F.);
#84734=ORIENTED_EDGE('',*,*,#57919,.T.);
#84735=ORIENTED_EDGE('',*,*,#53098,.F.);
#84736=ORIENTED_EDGE('',*,*,#57921,.F.);
#84737=ORIENTED_EDGE('',*,*,#56028,.F.);
#84738=ORIENTED_EDGE('',*,*,#57920,.T.);
#84739=ORIENTED_EDGE('',*,*,#56031,.F.);
#84740=ORIENTED_EDGE('',*,*,#57922,.F.);
#84741=ORIENTED_EDGE('',*,*,#53089,.F.);
#84742=ORIENTED_EDGE('',*,*,#57921,.T.);
#84743=ORIENTED_EDGE('',*,*,#53116,.F.);
#84744=ORIENTED_EDGE('',*,*,#57923,.F.);
#84745=ORIENTED_EDGE('',*,*,#56029,.F.);
#84746=ORIENTED_EDGE('',*,*,#57922,.T.);
#84747=ORIENTED_EDGE('',*,*,#56030,.F.);
#84748=ORIENTED_EDGE('',*,*,#57923,.T.);
#84749=ORIENTED_EDGE('',*,*,#53094,.F.);
#84750=ORIENTED_EDGE('',*,*,#53090,.T.);
#84751=ORIENTED_EDGE('',*,*,#57924,.F.);
#84752=ORIENTED_EDGE('',*,*,#56070,.F.);
#84753=ORIENTED_EDGE('',*,*,#57925,.F.);
#84754=ORIENTED_EDGE('',*,*,#53046,.F.);
#84755=ORIENTED_EDGE('',*,*,#57925,.T.);
#84756=ORIENTED_EDGE('',*,*,#56069,.F.);
#84757=ORIENTED_EDGE('',*,*,#57926,.F.);
#84758=ORIENTED_EDGE('',*,*,#53055,.F.);
#84759=ORIENTED_EDGE('',*,*,#53045,.T.);
#84760=ORIENTED_EDGE('',*,*,#53049,.F.);
#84761=ORIENTED_EDGE('',*,*,#57927,.F.);
#84762=ORIENTED_EDGE('',*,*,#56071,.F.);
#84763=ORIENTED_EDGE('',*,*,#57924,.T.);
#84764=ORIENTED_EDGE('',*,*,#57926,.T.);
#84765=ORIENTED_EDGE('',*,*,#56068,.F.);
#84766=ORIENTED_EDGE('',*,*,#57928,.F.);
#84767=ORIENTED_EDGE('',*,*,#53040,.F.);
#84768=ORIENTED_EDGE('',*,*,#57927,.T.);
#84769=ORIENTED_EDGE('',*,*,#53053,.F.);
#84770=ORIENTED_EDGE('',*,*,#57929,.F.);
#84771=ORIENTED_EDGE('',*,*,#56060,.F.);
#84772=ORIENTED_EDGE('',*,*,#57928,.T.);
#84773=ORIENTED_EDGE('',*,*,#56067,.F.);
#84774=ORIENTED_EDGE('',*,*,#57930,.F.);
#84775=ORIENTED_EDGE('',*,*,#53057,.F.);
#84776=ORIENTED_EDGE('',*,*,#57929,.T.);
#84777=ORIENTED_EDGE('',*,*,#52371,.F.);
#84778=ORIENTED_EDGE('',*,*,#57931,.F.);
#84779=ORIENTED_EDGE('',*,*,#56061,.F.);
#84780=ORIENTED_EDGE('',*,*,#57930,.T.);
#84781=ORIENTED_EDGE('',*,*,#56066,.F.);
#84782=ORIENTED_EDGE('',*,*,#57932,.F.);
#84783=ORIENTED_EDGE('',*,*,#53032,.T.);
#84784=ORIENTED_EDGE('',*,*,#53036,.F.);
#84785=ORIENTED_EDGE('',*,*,#57931,.T.);
#84786=ORIENTED_EDGE('',*,*,#52370,.F.);
#84787=ORIENTED_EDGE('',*,*,#57933,.F.);
#84788=ORIENTED_EDGE('',*,*,#56496,.F.);
#84789=ORIENTED_EDGE('',*,*,#57932,.T.);
#84790=ORIENTED_EDGE('',*,*,#56065,.F.);
#84791=ORIENTED_EDGE('',*,*,#57934,.F.);
#84792=ORIENTED_EDGE('',*,*,#53033,.F.);
#84793=ORIENTED_EDGE('',*,*,#57933,.T.);
#84794=ORIENTED_EDGE('',*,*,#52369,.F.);
#84795=ORIENTED_EDGE('',*,*,#57935,.F.);
#84796=ORIENTED_EDGE('',*,*,#56045,.F.);
#84797=ORIENTED_EDGE('',*,*,#57934,.T.);
#84798=ORIENTED_EDGE('',*,*,#56064,.F.);
#84799=ORIENTED_EDGE('',*,*,#57936,.F.);
#84800=ORIENTED_EDGE('',*,*,#53051,.F.);
#84801=ORIENTED_EDGE('',*,*,#57935,.T.);
#84802=ORIENTED_EDGE('',*,*,#52368,.F.);
#84803=ORIENTED_EDGE('',*,*,#57937,.F.);
#84804=ORIENTED_EDGE('',*,*,#56498,.F.);
#84805=ORIENTED_EDGE('',*,*,#57936,.T.);
#84806=ORIENTED_EDGE('',*,*,#56063,.F.);
#84807=ORIENTED_EDGE('',*,*,#57938,.F.);
#84808=ORIENTED_EDGE('',*,*,#52656,.F.);
#84809=ORIENTED_EDGE('',*,*,#57937,.T.);
#84810=ORIENTED_EDGE('',*,*,#52367,.F.);
#84811=ORIENTED_EDGE('',*,*,#57939,.F.);
#84812=ORIENTED_EDGE('',*,*,#56051,.F.);
#84813=ORIENTED_EDGE('',*,*,#57938,.T.);
#84814=ORIENTED_EDGE('',*,*,#56497,.F.);
#84815=ORIENTED_EDGE('',*,*,#57940,.F.);
#84816=ORIENTED_EDGE('',*,*,#52657,.F.);
#84817=ORIENTED_EDGE('',*,*,#57939,.T.);
#84818=ORIENTED_EDGE('',*,*,#53082,.F.);
#84819=ORIENTED_EDGE('',*,*,#57941,.F.);
#84820=ORIENTED_EDGE('',*,*,#56052,.F.);
#84821=ORIENTED_EDGE('',*,*,#57940,.T.);
#84822=ORIENTED_EDGE('',*,*,#56047,.F.);
#84823=ORIENTED_EDGE('',*,*,#57942,.F.);
#84824=ORIENTED_EDGE('',*,*,#52658,.F.);
#84825=ORIENTED_EDGE('',*,*,#53077,.F.);
#84826=ORIENTED_EDGE('',*,*,#53073,.T.);
#84827=ORIENTED_EDGE('',*,*,#57943,.F.);
#84828=ORIENTED_EDGE('',*,*,#56053,.F.);
#84829=ORIENTED_EDGE('',*,*,#57941,.T.);
#84830=ORIENTED_EDGE('',*,*,#57942,.T.);
#84831=ORIENTED_EDGE('',*,*,#56499,.F.);
#84832=ORIENTED_EDGE('',*,*,#57944,.F.);
#84833=ORIENTED_EDGE('',*,*,#52659,.F.);
#84834=ORIENTED_EDGE('',*,*,#57943,.T.);
#84835=ORIENTED_EDGE('',*,*,#53072,.F.);
#84836=ORIENTED_EDGE('',*,*,#57945,.F.);
#84837=ORIENTED_EDGE('',*,*,#56054,.F.);
#84838=ORIENTED_EDGE('',*,*,#57944,.T.);
#84839=ORIENTED_EDGE('',*,*,#56049,.F.);
#84840=ORIENTED_EDGE('',*,*,#57946,.F.);
#84841=ORIENTED_EDGE('',*,*,#52660,.F.);
#84842=ORIENTED_EDGE('',*,*,#57945,.T.);
#84843=ORIENTED_EDGE('',*,*,#53084,.F.);
#84844=ORIENTED_EDGE('',*,*,#57947,.F.);
#84845=ORIENTED_EDGE('',*,*,#56055,.F.);
#84846=ORIENTED_EDGE('',*,*,#57946,.T.);
#84847=ORIENTED_EDGE('',*,*,#56048,.F.);
#84848=ORIENTED_EDGE('',*,*,#57948,.F.);
#84849=ORIENTED_EDGE('',*,*,#53080,.F.);
#84850=ORIENTED_EDGE('',*,*,#57947,.T.);
#84851=ORIENTED_EDGE('',*,*,#53068,.F.);
#84852=ORIENTED_EDGE('',*,*,#57949,.F.);
#84853=ORIENTED_EDGE('',*,*,#56056,.F.);
#84854=ORIENTED_EDGE('',*,*,#57948,.T.);
#84855=ORIENTED_EDGE('',*,*,#56059,.F.);
#84856=ORIENTED_EDGE('',*,*,#57950,.F.);
#84857=ORIENTED_EDGE('',*,*,#53059,.F.);
#84858=ORIENTED_EDGE('',*,*,#57949,.T.);
#84859=ORIENTED_EDGE('',*,*,#53086,.F.);
#84860=ORIENTED_EDGE('',*,*,#57951,.F.);
#84861=ORIENTED_EDGE('',*,*,#56057,.F.);
#84862=ORIENTED_EDGE('',*,*,#57950,.T.);
#84863=ORIENTED_EDGE('',*,*,#56058,.F.);
#84864=ORIENTED_EDGE('',*,*,#57951,.T.);
#84865=ORIENTED_EDGE('',*,*,#53064,.F.);
#84866=ORIENTED_EDGE('',*,*,#53060,.T.);
#84867=ORIENTED_EDGE('',*,*,#57952,.F.);
#84868=ORIENTED_EDGE('',*,*,#56098,.F.);
#84869=ORIENTED_EDGE('',*,*,#57953,.F.);
#84870=ORIENTED_EDGE('',*,*,#53016,.F.);
#84871=ORIENTED_EDGE('',*,*,#57953,.T.);
#84872=ORIENTED_EDGE('',*,*,#56097,.F.);
#84873=ORIENTED_EDGE('',*,*,#57954,.F.);
#84874=ORIENTED_EDGE('',*,*,#53025,.F.);
#84875=ORIENTED_EDGE('',*,*,#53015,.T.);
#84876=ORIENTED_EDGE('',*,*,#53019,.F.);
#84877=ORIENTED_EDGE('',*,*,#57955,.F.);
#84878=ORIENTED_EDGE('',*,*,#56099,.F.);
#84879=ORIENTED_EDGE('',*,*,#57952,.T.);
#84880=ORIENTED_EDGE('',*,*,#57954,.T.);
#84881=ORIENTED_EDGE('',*,*,#56096,.F.);
#84882=ORIENTED_EDGE('',*,*,#57956,.F.);
#84883=ORIENTED_EDGE('',*,*,#53010,.F.);
#84884=ORIENTED_EDGE('',*,*,#57955,.T.);
#84885=ORIENTED_EDGE('',*,*,#53023,.F.);
#84886=ORIENTED_EDGE('',*,*,#57957,.F.);
#84887=ORIENTED_EDGE('',*,*,#56088,.F.);
#84888=ORIENTED_EDGE('',*,*,#57956,.T.);
#84889=ORIENTED_EDGE('',*,*,#56095,.F.);
#84890=ORIENTED_EDGE('',*,*,#57958,.F.);
#84891=ORIENTED_EDGE('',*,*,#53027,.F.);
#84892=ORIENTED_EDGE('',*,*,#57957,.T.);
#84893=ORIENTED_EDGE('',*,*,#52377,.F.);
#84894=ORIENTED_EDGE('',*,*,#57959,.F.);
#84895=ORIENTED_EDGE('',*,*,#56089,.F.);
#84896=ORIENTED_EDGE('',*,*,#57958,.T.);
#84897=ORIENTED_EDGE('',*,*,#56094,.F.);
#84898=ORIENTED_EDGE('',*,*,#57960,.F.);
#84899=ORIENTED_EDGE('',*,*,#53002,.T.);
#84900=ORIENTED_EDGE('',*,*,#53006,.F.);
#84901=ORIENTED_EDGE('',*,*,#57959,.T.);
#84902=ORIENTED_EDGE('',*,*,#52376,.F.);
#84903=ORIENTED_EDGE('',*,*,#57961,.F.);
#84904=ORIENTED_EDGE('',*,*,#56500,.F.);
#84905=ORIENTED_EDGE('',*,*,#57960,.T.);
#84906=ORIENTED_EDGE('',*,*,#56093,.F.);
#84907=ORIENTED_EDGE('',*,*,#57962,.F.);
#84908=ORIENTED_EDGE('',*,*,#53003,.F.);
#84909=ORIENTED_EDGE('',*,*,#57961,.T.);
#84910=ORIENTED_EDGE('',*,*,#52375,.F.);
#84911=ORIENTED_EDGE('',*,*,#57963,.F.);
#84912=ORIENTED_EDGE('',*,*,#56073,.F.);
#84913=ORIENTED_EDGE('',*,*,#57962,.T.);
#84914=ORIENTED_EDGE('',*,*,#56092,.F.);
#84915=ORIENTED_EDGE('',*,*,#57964,.F.);
#84916=ORIENTED_EDGE('',*,*,#53021,.F.);
#84917=ORIENTED_EDGE('',*,*,#57963,.T.);
#84918=ORIENTED_EDGE('',*,*,#52374,.F.);
#84919=ORIENTED_EDGE('',*,*,#57965,.F.);
#84920=ORIENTED_EDGE('',*,*,#56502,.F.);
#84921=ORIENTED_EDGE('',*,*,#57964,.T.);
#84922=ORIENTED_EDGE('',*,*,#56091,.F.);
#84923=ORIENTED_EDGE('',*,*,#57966,.F.);
#84924=ORIENTED_EDGE('',*,*,#52650,.F.);
#84925=ORIENTED_EDGE('',*,*,#57965,.T.);
#84926=ORIENTED_EDGE('',*,*,#52373,.F.);
#84927=ORIENTED_EDGE('',*,*,#57967,.F.);
#84928=ORIENTED_EDGE('',*,*,#56079,.F.);
#84929=ORIENTED_EDGE('',*,*,#57966,.T.);
#84930=ORIENTED_EDGE('',*,*,#56501,.F.);
#84931=ORIENTED_EDGE('',*,*,#57968,.F.);
#84932=ORIENTED_EDGE('',*,*,#52651,.F.);
#84933=ORIENTED_EDGE('',*,*,#57967,.T.);
#84934=ORIENTED_EDGE('',*,*,#53052,.F.);
#84935=ORIENTED_EDGE('',*,*,#57969,.F.);
#84936=ORIENTED_EDGE('',*,*,#56080,.F.);
#84937=ORIENTED_EDGE('',*,*,#57968,.T.);
#84938=ORIENTED_EDGE('',*,*,#56075,.F.);
#84939=ORIENTED_EDGE('',*,*,#57970,.F.);
#84940=ORIENTED_EDGE('',*,*,#52652,.F.);
#84941=ORIENTED_EDGE('',*,*,#53047,.F.);
#84942=ORIENTED_EDGE('',*,*,#53043,.T.);
#84943=ORIENTED_EDGE('',*,*,#57971,.F.);
#84944=ORIENTED_EDGE('',*,*,#56081,.F.);
#84945=ORIENTED_EDGE('',*,*,#57969,.T.);
#84946=ORIENTED_EDGE('',*,*,#57970,.T.);
#84947=ORIENTED_EDGE('',*,*,#56503,.F.);
#84948=ORIENTED_EDGE('',*,*,#57972,.F.);
#84949=ORIENTED_EDGE('',*,*,#52653,.F.);
#84950=ORIENTED_EDGE('',*,*,#57971,.T.);
#84951=ORIENTED_EDGE('',*,*,#53042,.F.);
#84952=ORIENTED_EDGE('',*,*,#57973,.F.);
#84953=ORIENTED_EDGE('',*,*,#56082,.F.);
#84954=ORIENTED_EDGE('',*,*,#57972,.T.);
#84955=ORIENTED_EDGE('',*,*,#56077,.F.);
#84956=ORIENTED_EDGE('',*,*,#57974,.F.);
#84957=ORIENTED_EDGE('',*,*,#52654,.F.);
#84958=ORIENTED_EDGE('',*,*,#57973,.T.);
#84959=ORIENTED_EDGE('',*,*,#53054,.F.);
#84960=ORIENTED_EDGE('',*,*,#57975,.F.);
#84961=ORIENTED_EDGE('',*,*,#56083,.F.);
#84962=ORIENTED_EDGE('',*,*,#57974,.T.);
#84963=ORIENTED_EDGE('',*,*,#56076,.F.);
#84964=ORIENTED_EDGE('',*,*,#57976,.F.);
#84965=ORIENTED_EDGE('',*,*,#53050,.F.);
#84966=ORIENTED_EDGE('',*,*,#57975,.T.);
#84967=ORIENTED_EDGE('',*,*,#53038,.F.);
#84968=ORIENTED_EDGE('',*,*,#57977,.F.);
#84969=ORIENTED_EDGE('',*,*,#56084,.F.);
#84970=ORIENTED_EDGE('',*,*,#57976,.T.);
#84971=ORIENTED_EDGE('',*,*,#56087,.F.);
#84972=ORIENTED_EDGE('',*,*,#57978,.F.);
#84973=ORIENTED_EDGE('',*,*,#53029,.F.);
#84974=ORIENTED_EDGE('',*,*,#57977,.T.);
#84975=ORIENTED_EDGE('',*,*,#53056,.F.);
#84976=ORIENTED_EDGE('',*,*,#57979,.F.);
#84977=ORIENTED_EDGE('',*,*,#56085,.F.);
#84978=ORIENTED_EDGE('',*,*,#57978,.T.);
#84979=ORIENTED_EDGE('',*,*,#56086,.F.);
#84980=ORIENTED_EDGE('',*,*,#57979,.T.);
#84981=ORIENTED_EDGE('',*,*,#53034,.F.);
#84982=ORIENTED_EDGE('',*,*,#53030,.T.);
#84983=ORIENTED_EDGE('',*,*,#57980,.F.);
#84984=ORIENTED_EDGE('',*,*,#56126,.F.);
#84985=ORIENTED_EDGE('',*,*,#57981,.F.);
#84986=ORIENTED_EDGE('',*,*,#52986,.F.);
#84987=ORIENTED_EDGE('',*,*,#57981,.T.);
#84988=ORIENTED_EDGE('',*,*,#56125,.F.);
#84989=ORIENTED_EDGE('',*,*,#57982,.F.);
#84990=ORIENTED_EDGE('',*,*,#52995,.F.);
#84991=ORIENTED_EDGE('',*,*,#52985,.T.);
#84992=ORIENTED_EDGE('',*,*,#52989,.F.);
#84993=ORIENTED_EDGE('',*,*,#57983,.F.);
#84994=ORIENTED_EDGE('',*,*,#56127,.F.);
#84995=ORIENTED_EDGE('',*,*,#57980,.T.);
#84996=ORIENTED_EDGE('',*,*,#57982,.T.);
#84997=ORIENTED_EDGE('',*,*,#56124,.F.);
#84998=ORIENTED_EDGE('',*,*,#57984,.F.);
#84999=ORIENTED_EDGE('',*,*,#52980,.F.);
#85000=ORIENTED_EDGE('',*,*,#57983,.T.);
#85001=ORIENTED_EDGE('',*,*,#52993,.F.);
#85002=ORIENTED_EDGE('',*,*,#57985,.F.);
#85003=ORIENTED_EDGE('',*,*,#56116,.F.);
#85004=ORIENTED_EDGE('',*,*,#57984,.T.);
#85005=ORIENTED_EDGE('',*,*,#56123,.F.);
#85006=ORIENTED_EDGE('',*,*,#57986,.F.);
#85007=ORIENTED_EDGE('',*,*,#52997,.F.);
#85008=ORIENTED_EDGE('',*,*,#57985,.T.);
#85009=ORIENTED_EDGE('',*,*,#52383,.F.);
#85010=ORIENTED_EDGE('',*,*,#57987,.F.);
#85011=ORIENTED_EDGE('',*,*,#56117,.F.);
#85012=ORIENTED_EDGE('',*,*,#57986,.T.);
#85013=ORIENTED_EDGE('',*,*,#56122,.F.);
#85014=ORIENTED_EDGE('',*,*,#57988,.F.);
#85015=ORIENTED_EDGE('',*,*,#52972,.T.);
#85016=ORIENTED_EDGE('',*,*,#52976,.F.);
#85017=ORIENTED_EDGE('',*,*,#57987,.T.);
#85018=ORIENTED_EDGE('',*,*,#52382,.F.);
#85019=ORIENTED_EDGE('',*,*,#57989,.F.);
#85020=ORIENTED_EDGE('',*,*,#56504,.F.);
#85021=ORIENTED_EDGE('',*,*,#57988,.T.);
#85022=ORIENTED_EDGE('',*,*,#56121,.F.);
#85023=ORIENTED_EDGE('',*,*,#57990,.F.);
#85024=ORIENTED_EDGE('',*,*,#52973,.F.);
#85025=ORIENTED_EDGE('',*,*,#57989,.T.);
#85026=ORIENTED_EDGE('',*,*,#52381,.F.);
#85027=ORIENTED_EDGE('',*,*,#57991,.F.);
#85028=ORIENTED_EDGE('',*,*,#56101,.F.);
#85029=ORIENTED_EDGE('',*,*,#57990,.T.);
#85030=ORIENTED_EDGE('',*,*,#56120,.F.);
#85031=ORIENTED_EDGE('',*,*,#57992,.F.);
#85032=ORIENTED_EDGE('',*,*,#52991,.F.);
#85033=ORIENTED_EDGE('',*,*,#57991,.T.);
#85034=ORIENTED_EDGE('',*,*,#52380,.F.);
#85035=ORIENTED_EDGE('',*,*,#57993,.F.);
#85036=ORIENTED_EDGE('',*,*,#56506,.F.);
#85037=ORIENTED_EDGE('',*,*,#57992,.T.);
#85038=ORIENTED_EDGE('',*,*,#56119,.F.);
#85039=ORIENTED_EDGE('',*,*,#57994,.F.);
#85040=ORIENTED_EDGE('',*,*,#52644,.F.);
#85041=ORIENTED_EDGE('',*,*,#57993,.T.);
#85042=ORIENTED_EDGE('',*,*,#52379,.F.);
#85043=ORIENTED_EDGE('',*,*,#57995,.F.);
#85044=ORIENTED_EDGE('',*,*,#56107,.F.);
#85045=ORIENTED_EDGE('',*,*,#57994,.T.);
#85046=ORIENTED_EDGE('',*,*,#56505,.F.);
#85047=ORIENTED_EDGE('',*,*,#57996,.F.);
#85048=ORIENTED_EDGE('',*,*,#52645,.F.);
#85049=ORIENTED_EDGE('',*,*,#57995,.T.);
#85050=ORIENTED_EDGE('',*,*,#53022,.F.);
#85051=ORIENTED_EDGE('',*,*,#57997,.F.);
#85052=ORIENTED_EDGE('',*,*,#56108,.F.);
#85053=ORIENTED_EDGE('',*,*,#57996,.T.);
#85054=ORIENTED_EDGE('',*,*,#56103,.F.);
#85055=ORIENTED_EDGE('',*,*,#57998,.F.);
#85056=ORIENTED_EDGE('',*,*,#52646,.F.);
#85057=ORIENTED_EDGE('',*,*,#53017,.F.);
#85058=ORIENTED_EDGE('',*,*,#53013,.T.);
#85059=ORIENTED_EDGE('',*,*,#57999,.F.);
#85060=ORIENTED_EDGE('',*,*,#56109,.F.);
#85061=ORIENTED_EDGE('',*,*,#57997,.T.);
#85062=ORIENTED_EDGE('',*,*,#57998,.T.);
#85063=ORIENTED_EDGE('',*,*,#56507,.F.);
#85064=ORIENTED_EDGE('',*,*,#58000,.F.);
#85065=ORIENTED_EDGE('',*,*,#52647,.F.);
#85066=ORIENTED_EDGE('',*,*,#57999,.T.);
#85067=ORIENTED_EDGE('',*,*,#53012,.F.);
#85068=ORIENTED_EDGE('',*,*,#58001,.F.);
#85069=ORIENTED_EDGE('',*,*,#56110,.F.);
#85070=ORIENTED_EDGE('',*,*,#58000,.T.);
#85071=ORIENTED_EDGE('',*,*,#56105,.F.);
#85072=ORIENTED_EDGE('',*,*,#58002,.F.);
#85073=ORIENTED_EDGE('',*,*,#52648,.F.);
#85074=ORIENTED_EDGE('',*,*,#58001,.T.);
#85075=ORIENTED_EDGE('',*,*,#53024,.F.);
#85076=ORIENTED_EDGE('',*,*,#58003,.F.);
#85077=ORIENTED_EDGE('',*,*,#56111,.F.);
#85078=ORIENTED_EDGE('',*,*,#58002,.T.);
#85079=ORIENTED_EDGE('',*,*,#56104,.F.);
#85080=ORIENTED_EDGE('',*,*,#58004,.F.);
#85081=ORIENTED_EDGE('',*,*,#53020,.F.);
#85082=ORIENTED_EDGE('',*,*,#58003,.T.);
#85083=ORIENTED_EDGE('',*,*,#53008,.F.);
#85084=ORIENTED_EDGE('',*,*,#58005,.F.);
#85085=ORIENTED_EDGE('',*,*,#56112,.F.);
#85086=ORIENTED_EDGE('',*,*,#58004,.T.);
#85087=ORIENTED_EDGE('',*,*,#56115,.F.);
#85088=ORIENTED_EDGE('',*,*,#58006,.F.);
#85089=ORIENTED_EDGE('',*,*,#52999,.F.);
#85090=ORIENTED_EDGE('',*,*,#58005,.T.);
#85091=ORIENTED_EDGE('',*,*,#53026,.F.);
#85092=ORIENTED_EDGE('',*,*,#58007,.F.);
#85093=ORIENTED_EDGE('',*,*,#56113,.F.);
#85094=ORIENTED_EDGE('',*,*,#58006,.T.);
#85095=ORIENTED_EDGE('',*,*,#56114,.F.);
#85096=ORIENTED_EDGE('',*,*,#58007,.T.);
#85097=ORIENTED_EDGE('',*,*,#53004,.F.);
#85098=ORIENTED_EDGE('',*,*,#53000,.T.);
#85099=ORIENTED_EDGE('',*,*,#58008,.F.);
#85100=ORIENTED_EDGE('',*,*,#56154,.F.);
#85101=ORIENTED_EDGE('',*,*,#58009,.F.);
#85102=ORIENTED_EDGE('',*,*,#52956,.F.);
#85103=ORIENTED_EDGE('',*,*,#58009,.T.);
#85104=ORIENTED_EDGE('',*,*,#56153,.F.);
#85105=ORIENTED_EDGE('',*,*,#58010,.F.);
#85106=ORIENTED_EDGE('',*,*,#52965,.F.);
#85107=ORIENTED_EDGE('',*,*,#52955,.T.);
#85108=ORIENTED_EDGE('',*,*,#52959,.F.);
#85109=ORIENTED_EDGE('',*,*,#58011,.F.);
#85110=ORIENTED_EDGE('',*,*,#56155,.F.);
#85111=ORIENTED_EDGE('',*,*,#58008,.T.);
#85112=ORIENTED_EDGE('',*,*,#58010,.T.);
#85113=ORIENTED_EDGE('',*,*,#56152,.F.);
#85114=ORIENTED_EDGE('',*,*,#58012,.F.);
#85115=ORIENTED_EDGE('',*,*,#52950,.F.);
#85116=ORIENTED_EDGE('',*,*,#58011,.T.);
#85117=ORIENTED_EDGE('',*,*,#52963,.F.);
#85118=ORIENTED_EDGE('',*,*,#58013,.F.);
#85119=ORIENTED_EDGE('',*,*,#56144,.F.);
#85120=ORIENTED_EDGE('',*,*,#58012,.T.);
#85121=ORIENTED_EDGE('',*,*,#56151,.F.);
#85122=ORIENTED_EDGE('',*,*,#58014,.F.);
#85123=ORIENTED_EDGE('',*,*,#52967,.F.);
#85124=ORIENTED_EDGE('',*,*,#58013,.T.);
#85125=ORIENTED_EDGE('',*,*,#52389,.F.);
#85126=ORIENTED_EDGE('',*,*,#58015,.F.);
#85127=ORIENTED_EDGE('',*,*,#56145,.F.);
#85128=ORIENTED_EDGE('',*,*,#58014,.T.);
#85129=ORIENTED_EDGE('',*,*,#56150,.F.);
#85130=ORIENTED_EDGE('',*,*,#58016,.F.);
#85131=ORIENTED_EDGE('',*,*,#52942,.T.);
#85132=ORIENTED_EDGE('',*,*,#52946,.F.);
#85133=ORIENTED_EDGE('',*,*,#58015,.T.);
#85134=ORIENTED_EDGE('',*,*,#52388,.F.);
#85135=ORIENTED_EDGE('',*,*,#58017,.F.);
#85136=ORIENTED_EDGE('',*,*,#56508,.F.);
#85137=ORIENTED_EDGE('',*,*,#58016,.T.);
#85138=ORIENTED_EDGE('',*,*,#56149,.F.);
#85139=ORIENTED_EDGE('',*,*,#58018,.F.);
#85140=ORIENTED_EDGE('',*,*,#52943,.F.);
#85141=ORIENTED_EDGE('',*,*,#58017,.T.);
#85142=ORIENTED_EDGE('',*,*,#52387,.F.);
#85143=ORIENTED_EDGE('',*,*,#58019,.F.);
#85144=ORIENTED_EDGE('',*,*,#56129,.F.);
#85145=ORIENTED_EDGE('',*,*,#58018,.T.);
#85146=ORIENTED_EDGE('',*,*,#56148,.F.);
#85147=ORIENTED_EDGE('',*,*,#58020,.F.);
#85148=ORIENTED_EDGE('',*,*,#52961,.F.);
#85149=ORIENTED_EDGE('',*,*,#58019,.T.);
#85150=ORIENTED_EDGE('',*,*,#52386,.F.);
#85151=ORIENTED_EDGE('',*,*,#58021,.F.);
#85152=ORIENTED_EDGE('',*,*,#56510,.F.);
#85153=ORIENTED_EDGE('',*,*,#58020,.T.);
#85154=ORIENTED_EDGE('',*,*,#56147,.F.);
#85155=ORIENTED_EDGE('',*,*,#58022,.F.);
#85156=ORIENTED_EDGE('',*,*,#52638,.F.);
#85157=ORIENTED_EDGE('',*,*,#58021,.T.);
#85158=ORIENTED_EDGE('',*,*,#52385,.F.);
#85159=ORIENTED_EDGE('',*,*,#58023,.F.);
#85160=ORIENTED_EDGE('',*,*,#56135,.F.);
#85161=ORIENTED_EDGE('',*,*,#58022,.T.);
#85162=ORIENTED_EDGE('',*,*,#56509,.F.);
#85163=ORIENTED_EDGE('',*,*,#58024,.F.);
#85164=ORIENTED_EDGE('',*,*,#52639,.F.);
#85165=ORIENTED_EDGE('',*,*,#58023,.T.);
#85166=ORIENTED_EDGE('',*,*,#52992,.F.);
#85167=ORIENTED_EDGE('',*,*,#58025,.F.);
#85168=ORIENTED_EDGE('',*,*,#56136,.F.);
#85169=ORIENTED_EDGE('',*,*,#58024,.T.);
#85170=ORIENTED_EDGE('',*,*,#56131,.F.);
#85171=ORIENTED_EDGE('',*,*,#58026,.F.);
#85172=ORIENTED_EDGE('',*,*,#52640,.F.);
#85173=ORIENTED_EDGE('',*,*,#52987,.F.);
#85174=ORIENTED_EDGE('',*,*,#52983,.T.);
#85175=ORIENTED_EDGE('',*,*,#58027,.F.);
#85176=ORIENTED_EDGE('',*,*,#56137,.F.);
#85177=ORIENTED_EDGE('',*,*,#58025,.T.);
#85178=ORIENTED_EDGE('',*,*,#58026,.T.);
#85179=ORIENTED_EDGE('',*,*,#56511,.F.);
#85180=ORIENTED_EDGE('',*,*,#58028,.F.);
#85181=ORIENTED_EDGE('',*,*,#52641,.F.);
#85182=ORIENTED_EDGE('',*,*,#58027,.T.);
#85183=ORIENTED_EDGE('',*,*,#52982,.F.);
#85184=ORIENTED_EDGE('',*,*,#58029,.F.);
#85185=ORIENTED_EDGE('',*,*,#56138,.F.);
#85186=ORIENTED_EDGE('',*,*,#58028,.T.);
#85187=ORIENTED_EDGE('',*,*,#56133,.F.);
#85188=ORIENTED_EDGE('',*,*,#58030,.F.);
#85189=ORIENTED_EDGE('',*,*,#52642,.F.);
#85190=ORIENTED_EDGE('',*,*,#58029,.T.);
#85191=ORIENTED_EDGE('',*,*,#52994,.F.);
#85192=ORIENTED_EDGE('',*,*,#58031,.F.);
#85193=ORIENTED_EDGE('',*,*,#56139,.F.);
#85194=ORIENTED_EDGE('',*,*,#58030,.T.);
#85195=ORIENTED_EDGE('',*,*,#56132,.F.);
#85196=ORIENTED_EDGE('',*,*,#58032,.F.);
#85197=ORIENTED_EDGE('',*,*,#52990,.F.);
#85198=ORIENTED_EDGE('',*,*,#58031,.T.);
#85199=ORIENTED_EDGE('',*,*,#52978,.F.);
#85200=ORIENTED_EDGE('',*,*,#58033,.F.);
#85201=ORIENTED_EDGE('',*,*,#56140,.F.);
#85202=ORIENTED_EDGE('',*,*,#58032,.T.);
#85203=ORIENTED_EDGE('',*,*,#56143,.F.);
#85204=ORIENTED_EDGE('',*,*,#58034,.F.);
#85205=ORIENTED_EDGE('',*,*,#52969,.F.);
#85206=ORIENTED_EDGE('',*,*,#58033,.T.);
#85207=ORIENTED_EDGE('',*,*,#52996,.F.);
#85208=ORIENTED_EDGE('',*,*,#58035,.F.);
#85209=ORIENTED_EDGE('',*,*,#56141,.F.);
#85210=ORIENTED_EDGE('',*,*,#58034,.T.);
#85211=ORIENTED_EDGE('',*,*,#56142,.F.);
#85212=ORIENTED_EDGE('',*,*,#58035,.T.);
#85213=ORIENTED_EDGE('',*,*,#52974,.F.);
#85214=ORIENTED_EDGE('',*,*,#52970,.T.);
#85215=ORIENTED_EDGE('',*,*,#58036,.F.);
#85216=ORIENTED_EDGE('',*,*,#56182,.F.);
#85217=ORIENTED_EDGE('',*,*,#58037,.F.);
#85218=ORIENTED_EDGE('',*,*,#52926,.F.);
#85219=ORIENTED_EDGE('',*,*,#58037,.T.);
#85220=ORIENTED_EDGE('',*,*,#56181,.F.);
#85221=ORIENTED_EDGE('',*,*,#58038,.F.);
#85222=ORIENTED_EDGE('',*,*,#52935,.F.);
#85223=ORIENTED_EDGE('',*,*,#52925,.T.);
#85224=ORIENTED_EDGE('',*,*,#52929,.F.);
#85225=ORIENTED_EDGE('',*,*,#58039,.F.);
#85226=ORIENTED_EDGE('',*,*,#56183,.F.);
#85227=ORIENTED_EDGE('',*,*,#58036,.T.);
#85228=ORIENTED_EDGE('',*,*,#58038,.T.);
#85229=ORIENTED_EDGE('',*,*,#56180,.F.);
#85230=ORIENTED_EDGE('',*,*,#58040,.F.);
#85231=ORIENTED_EDGE('',*,*,#52920,.F.);
#85232=ORIENTED_EDGE('',*,*,#58039,.T.);
#85233=ORIENTED_EDGE('',*,*,#52933,.F.);
#85234=ORIENTED_EDGE('',*,*,#58041,.F.);
#85235=ORIENTED_EDGE('',*,*,#56172,.F.);
#85236=ORIENTED_EDGE('',*,*,#58040,.T.);
#85237=ORIENTED_EDGE('',*,*,#56179,.F.);
#85238=ORIENTED_EDGE('',*,*,#58042,.F.);
#85239=ORIENTED_EDGE('',*,*,#52937,.F.);
#85240=ORIENTED_EDGE('',*,*,#58041,.T.);
#85241=ORIENTED_EDGE('',*,*,#52395,.F.);
#85242=ORIENTED_EDGE('',*,*,#58043,.F.);
#85243=ORIENTED_EDGE('',*,*,#56173,.F.);
#85244=ORIENTED_EDGE('',*,*,#58042,.T.);
#85245=ORIENTED_EDGE('',*,*,#56178,.F.);
#85246=ORIENTED_EDGE('',*,*,#58044,.F.);
#85247=ORIENTED_EDGE('',*,*,#52912,.T.);
#85248=ORIENTED_EDGE('',*,*,#52916,.F.);
#85249=ORIENTED_EDGE('',*,*,#58043,.T.);
#85250=ORIENTED_EDGE('',*,*,#52394,.F.);
#85251=ORIENTED_EDGE('',*,*,#58045,.F.);
#85252=ORIENTED_EDGE('',*,*,#56512,.F.);
#85253=ORIENTED_EDGE('',*,*,#58044,.T.);
#85254=ORIENTED_EDGE('',*,*,#56177,.F.);
#85255=ORIENTED_EDGE('',*,*,#58046,.F.);
#85256=ORIENTED_EDGE('',*,*,#52913,.F.);
#85257=ORIENTED_EDGE('',*,*,#58045,.T.);
#85258=ORIENTED_EDGE('',*,*,#52393,.F.);
#85259=ORIENTED_EDGE('',*,*,#58047,.F.);
#85260=ORIENTED_EDGE('',*,*,#56157,.F.);
#85261=ORIENTED_EDGE('',*,*,#58046,.T.);
#85262=ORIENTED_EDGE('',*,*,#56176,.F.);
#85263=ORIENTED_EDGE('',*,*,#58048,.F.);
#85264=ORIENTED_EDGE('',*,*,#52931,.F.);
#85265=ORIENTED_EDGE('',*,*,#58047,.T.);
#85266=ORIENTED_EDGE('',*,*,#52392,.F.);
#85267=ORIENTED_EDGE('',*,*,#58049,.F.);
#85268=ORIENTED_EDGE('',*,*,#56514,.F.);
#85269=ORIENTED_EDGE('',*,*,#58048,.T.);
#85270=ORIENTED_EDGE('',*,*,#56175,.F.);
#85271=ORIENTED_EDGE('',*,*,#58050,.F.);
#85272=ORIENTED_EDGE('',*,*,#52632,.F.);
#85273=ORIENTED_EDGE('',*,*,#58049,.T.);
#85274=ORIENTED_EDGE('',*,*,#52391,.F.);
#85275=ORIENTED_EDGE('',*,*,#58051,.F.);
#85276=ORIENTED_EDGE('',*,*,#56163,.F.);
#85277=ORIENTED_EDGE('',*,*,#58050,.T.);
#85278=ORIENTED_EDGE('',*,*,#56513,.F.);
#85279=ORIENTED_EDGE('',*,*,#58052,.F.);
#85280=ORIENTED_EDGE('',*,*,#52633,.F.);
#85281=ORIENTED_EDGE('',*,*,#58051,.T.);
#85282=ORIENTED_EDGE('',*,*,#52962,.F.);
#85283=ORIENTED_EDGE('',*,*,#58053,.F.);
#85284=ORIENTED_EDGE('',*,*,#56164,.F.);
#85285=ORIENTED_EDGE('',*,*,#58052,.T.);
#85286=ORIENTED_EDGE('',*,*,#56159,.F.);
#85287=ORIENTED_EDGE('',*,*,#58054,.F.);
#85288=ORIENTED_EDGE('',*,*,#52634,.F.);
#85289=ORIENTED_EDGE('',*,*,#52957,.F.);
#85290=ORIENTED_EDGE('',*,*,#52953,.T.);
#85291=ORIENTED_EDGE('',*,*,#58055,.F.);
#85292=ORIENTED_EDGE('',*,*,#56165,.F.);
#85293=ORIENTED_EDGE('',*,*,#58053,.T.);
#85294=ORIENTED_EDGE('',*,*,#58054,.T.);
#85295=ORIENTED_EDGE('',*,*,#56515,.F.);
#85296=ORIENTED_EDGE('',*,*,#58056,.F.);
#85297=ORIENTED_EDGE('',*,*,#52635,.F.);
#85298=ORIENTED_EDGE('',*,*,#58055,.T.);
#85299=ORIENTED_EDGE('',*,*,#52952,.F.);
#85300=ORIENTED_EDGE('',*,*,#58057,.F.);
#85301=ORIENTED_EDGE('',*,*,#56166,.F.);
#85302=ORIENTED_EDGE('',*,*,#58056,.T.);
#85303=ORIENTED_EDGE('',*,*,#56161,.F.);
#85304=ORIENTED_EDGE('',*,*,#58058,.F.);
#85305=ORIENTED_EDGE('',*,*,#52636,.F.);
#85306=ORIENTED_EDGE('',*,*,#58057,.T.);
#85307=ORIENTED_EDGE('',*,*,#52964,.F.);
#85308=ORIENTED_EDGE('',*,*,#58059,.F.);
#85309=ORIENTED_EDGE('',*,*,#56167,.F.);
#85310=ORIENTED_EDGE('',*,*,#58058,.T.);
#85311=ORIENTED_EDGE('',*,*,#56160,.F.);
#85312=ORIENTED_EDGE('',*,*,#58060,.F.);
#85313=ORIENTED_EDGE('',*,*,#52960,.F.);
#85314=ORIENTED_EDGE('',*,*,#58059,.T.);
#85315=ORIENTED_EDGE('',*,*,#52948,.F.);
#85316=ORIENTED_EDGE('',*,*,#58061,.F.);
#85317=ORIENTED_EDGE('',*,*,#56168,.F.);
#85318=ORIENTED_EDGE('',*,*,#58060,.T.);
#85319=ORIENTED_EDGE('',*,*,#56171,.F.);
#85320=ORIENTED_EDGE('',*,*,#58062,.F.);
#85321=ORIENTED_EDGE('',*,*,#52939,.F.);
#85322=ORIENTED_EDGE('',*,*,#58061,.T.);
#85323=ORIENTED_EDGE('',*,*,#52966,.F.);
#85324=ORIENTED_EDGE('',*,*,#58063,.F.);
#85325=ORIENTED_EDGE('',*,*,#56169,.F.);
#85326=ORIENTED_EDGE('',*,*,#58062,.T.);
#85327=ORIENTED_EDGE('',*,*,#56170,.F.);
#85328=ORIENTED_EDGE('',*,*,#58063,.T.);
#85329=ORIENTED_EDGE('',*,*,#52944,.F.);
#85330=ORIENTED_EDGE('',*,*,#52940,.T.);
#85331=ORIENTED_EDGE('',*,*,#58064,.F.);
#85332=ORIENTED_EDGE('',*,*,#56210,.F.);
#85333=ORIENTED_EDGE('',*,*,#58065,.F.);
#85334=ORIENTED_EDGE('',*,*,#52896,.F.);
#85335=ORIENTED_EDGE('',*,*,#58065,.T.);
#85336=ORIENTED_EDGE('',*,*,#56209,.F.);
#85337=ORIENTED_EDGE('',*,*,#58066,.F.);
#85338=ORIENTED_EDGE('',*,*,#52905,.F.);
#85339=ORIENTED_EDGE('',*,*,#52895,.T.);
#85340=ORIENTED_EDGE('',*,*,#52899,.F.);
#85341=ORIENTED_EDGE('',*,*,#58067,.F.);
#85342=ORIENTED_EDGE('',*,*,#56211,.F.);
#85343=ORIENTED_EDGE('',*,*,#58064,.T.);
#85344=ORIENTED_EDGE('',*,*,#58066,.T.);
#85345=ORIENTED_EDGE('',*,*,#56208,.F.);
#85346=ORIENTED_EDGE('',*,*,#58068,.F.);
#85347=ORIENTED_EDGE('',*,*,#52890,.F.);
#85348=ORIENTED_EDGE('',*,*,#58067,.T.);
#85349=ORIENTED_EDGE('',*,*,#52903,.F.);
#85350=ORIENTED_EDGE('',*,*,#58069,.F.);
#85351=ORIENTED_EDGE('',*,*,#56200,.F.);
#85352=ORIENTED_EDGE('',*,*,#58068,.T.);
#85353=ORIENTED_EDGE('',*,*,#56207,.F.);
#85354=ORIENTED_EDGE('',*,*,#58070,.F.);
#85355=ORIENTED_EDGE('',*,*,#52907,.F.);
#85356=ORIENTED_EDGE('',*,*,#58069,.T.);
#85357=ORIENTED_EDGE('',*,*,#52401,.F.);
#85358=ORIENTED_EDGE('',*,*,#58071,.F.);
#85359=ORIENTED_EDGE('',*,*,#56201,.F.);
#85360=ORIENTED_EDGE('',*,*,#58070,.T.);
#85361=ORIENTED_EDGE('',*,*,#56206,.F.);
#85362=ORIENTED_EDGE('',*,*,#58072,.F.);
#85363=ORIENTED_EDGE('',*,*,#52882,.T.);
#85364=ORIENTED_EDGE('',*,*,#52886,.F.);
#85365=ORIENTED_EDGE('',*,*,#58071,.T.);
#85366=ORIENTED_EDGE('',*,*,#52400,.F.);
#85367=ORIENTED_EDGE('',*,*,#58073,.F.);
#85368=ORIENTED_EDGE('',*,*,#56516,.F.);
#85369=ORIENTED_EDGE('',*,*,#58072,.T.);
#85370=ORIENTED_EDGE('',*,*,#56205,.F.);
#85371=ORIENTED_EDGE('',*,*,#58074,.F.);
#85372=ORIENTED_EDGE('',*,*,#52883,.F.);
#85373=ORIENTED_EDGE('',*,*,#58073,.T.);
#85374=ORIENTED_EDGE('',*,*,#52399,.F.);
#85375=ORIENTED_EDGE('',*,*,#58075,.F.);
#85376=ORIENTED_EDGE('',*,*,#56185,.F.);
#85377=ORIENTED_EDGE('',*,*,#58074,.T.);
#85378=ORIENTED_EDGE('',*,*,#56204,.F.);
#85379=ORIENTED_EDGE('',*,*,#58076,.F.);
#85380=ORIENTED_EDGE('',*,*,#52901,.F.);
#85381=ORIENTED_EDGE('',*,*,#58075,.T.);
#85382=ORIENTED_EDGE('',*,*,#52398,.F.);
#85383=ORIENTED_EDGE('',*,*,#58077,.F.);
#85384=ORIENTED_EDGE('',*,*,#56518,.F.);
#85385=ORIENTED_EDGE('',*,*,#58076,.T.);
#85386=ORIENTED_EDGE('',*,*,#56203,.F.);
#85387=ORIENTED_EDGE('',*,*,#58078,.F.);
#85388=ORIENTED_EDGE('',*,*,#52626,.F.);
#85389=ORIENTED_EDGE('',*,*,#58077,.T.);
#85390=ORIENTED_EDGE('',*,*,#52397,.F.);
#85391=ORIENTED_EDGE('',*,*,#58079,.F.);
#85392=ORIENTED_EDGE('',*,*,#56191,.F.);
#85393=ORIENTED_EDGE('',*,*,#58078,.T.);
#85394=ORIENTED_EDGE('',*,*,#56517,.F.);
#85395=ORIENTED_EDGE('',*,*,#58080,.F.);
#85396=ORIENTED_EDGE('',*,*,#52627,.F.);
#85397=ORIENTED_EDGE('',*,*,#58079,.T.);
#85398=ORIENTED_EDGE('',*,*,#52932,.F.);
#85399=ORIENTED_EDGE('',*,*,#58081,.F.);
#85400=ORIENTED_EDGE('',*,*,#56192,.F.);
#85401=ORIENTED_EDGE('',*,*,#58080,.T.);
#85402=ORIENTED_EDGE('',*,*,#56187,.F.);
#85403=ORIENTED_EDGE('',*,*,#58082,.F.);
#85404=ORIENTED_EDGE('',*,*,#52628,.F.);
#85405=ORIENTED_EDGE('',*,*,#52927,.F.);
#85406=ORIENTED_EDGE('',*,*,#52923,.T.);
#85407=ORIENTED_EDGE('',*,*,#58083,.F.);
#85408=ORIENTED_EDGE('',*,*,#56193,.F.);
#85409=ORIENTED_EDGE('',*,*,#58081,.T.);
#85410=ORIENTED_EDGE('',*,*,#58082,.T.);
#85411=ORIENTED_EDGE('',*,*,#56519,.F.);
#85412=ORIENTED_EDGE('',*,*,#58084,.F.);
#85413=ORIENTED_EDGE('',*,*,#52629,.F.);
#85414=ORIENTED_EDGE('',*,*,#58083,.T.);
#85415=ORIENTED_EDGE('',*,*,#52922,.F.);
#85416=ORIENTED_EDGE('',*,*,#58085,.F.);
#85417=ORIENTED_EDGE('',*,*,#56194,.F.);
#85418=ORIENTED_EDGE('',*,*,#58084,.T.);
#85419=ORIENTED_EDGE('',*,*,#56189,.F.);
#85420=ORIENTED_EDGE('',*,*,#58086,.F.);
#85421=ORIENTED_EDGE('',*,*,#52630,.F.);
#85422=ORIENTED_EDGE('',*,*,#58085,.T.);
#85423=ORIENTED_EDGE('',*,*,#52934,.F.);
#85424=ORIENTED_EDGE('',*,*,#58087,.F.);
#85425=ORIENTED_EDGE('',*,*,#56195,.F.);
#85426=ORIENTED_EDGE('',*,*,#58086,.T.);
#85427=ORIENTED_EDGE('',*,*,#56188,.F.);
#85428=ORIENTED_EDGE('',*,*,#58088,.F.);
#85429=ORIENTED_EDGE('',*,*,#52930,.F.);
#85430=ORIENTED_EDGE('',*,*,#58087,.T.);
#85431=ORIENTED_EDGE('',*,*,#52918,.F.);
#85432=ORIENTED_EDGE('',*,*,#58089,.F.);
#85433=ORIENTED_EDGE('',*,*,#56196,.F.);
#85434=ORIENTED_EDGE('',*,*,#58088,.T.);
#85435=ORIENTED_EDGE('',*,*,#56199,.F.);
#85436=ORIENTED_EDGE('',*,*,#58090,.F.);
#85437=ORIENTED_EDGE('',*,*,#52909,.F.);
#85438=ORIENTED_EDGE('',*,*,#58089,.T.);
#85439=ORIENTED_EDGE('',*,*,#52936,.F.);
#85440=ORIENTED_EDGE('',*,*,#58091,.F.);
#85441=ORIENTED_EDGE('',*,*,#56197,.F.);
#85442=ORIENTED_EDGE('',*,*,#58090,.T.);
#85443=ORIENTED_EDGE('',*,*,#56198,.F.);
#85444=ORIENTED_EDGE('',*,*,#58091,.T.);
#85445=ORIENTED_EDGE('',*,*,#52914,.F.);
#85446=ORIENTED_EDGE('',*,*,#52910,.T.);
#85447=ORIENTED_EDGE('',*,*,#58092,.F.);
#85448=ORIENTED_EDGE('',*,*,#56238,.F.);
#85449=ORIENTED_EDGE('',*,*,#58093,.F.);
#85450=ORIENTED_EDGE('',*,*,#52866,.F.);
#85451=ORIENTED_EDGE('',*,*,#58093,.T.);
#85452=ORIENTED_EDGE('',*,*,#56237,.F.);
#85453=ORIENTED_EDGE('',*,*,#58094,.F.);
#85454=ORIENTED_EDGE('',*,*,#52875,.F.);
#85455=ORIENTED_EDGE('',*,*,#52865,.T.);
#85456=ORIENTED_EDGE('',*,*,#52869,.F.);
#85457=ORIENTED_EDGE('',*,*,#58095,.F.);
#85458=ORIENTED_EDGE('',*,*,#56239,.F.);
#85459=ORIENTED_EDGE('',*,*,#58092,.T.);
#85460=ORIENTED_EDGE('',*,*,#58094,.T.);
#85461=ORIENTED_EDGE('',*,*,#56236,.F.);
#85462=ORIENTED_EDGE('',*,*,#58096,.F.);
#85463=ORIENTED_EDGE('',*,*,#52860,.F.);
#85464=ORIENTED_EDGE('',*,*,#58095,.T.);
#85465=ORIENTED_EDGE('',*,*,#52873,.F.);
#85466=ORIENTED_EDGE('',*,*,#58097,.F.);
#85467=ORIENTED_EDGE('',*,*,#56228,.F.);
#85468=ORIENTED_EDGE('',*,*,#58096,.T.);
#85469=ORIENTED_EDGE('',*,*,#56235,.F.);
#85470=ORIENTED_EDGE('',*,*,#58098,.F.);
#85471=ORIENTED_EDGE('',*,*,#52877,.F.);
#85472=ORIENTED_EDGE('',*,*,#58097,.T.);
#85473=ORIENTED_EDGE('',*,*,#52407,.F.);
#85474=ORIENTED_EDGE('',*,*,#58099,.F.);
#85475=ORIENTED_EDGE('',*,*,#56229,.F.);
#85476=ORIENTED_EDGE('',*,*,#58098,.T.);
#85477=ORIENTED_EDGE('',*,*,#56234,.F.);
#85478=ORIENTED_EDGE('',*,*,#58100,.F.);
#85479=ORIENTED_EDGE('',*,*,#52852,.T.);
#85480=ORIENTED_EDGE('',*,*,#52856,.F.);
#85481=ORIENTED_EDGE('',*,*,#58099,.T.);
#85482=ORIENTED_EDGE('',*,*,#52406,.F.);
#85483=ORIENTED_EDGE('',*,*,#58101,.F.);
#85484=ORIENTED_EDGE('',*,*,#56520,.F.);
#85485=ORIENTED_EDGE('',*,*,#58100,.T.);
#85486=ORIENTED_EDGE('',*,*,#56233,.F.);
#85487=ORIENTED_EDGE('',*,*,#58102,.F.);
#85488=ORIENTED_EDGE('',*,*,#52853,.F.);
#85489=ORIENTED_EDGE('',*,*,#58101,.T.);
#85490=ORIENTED_EDGE('',*,*,#52405,.F.);
#85491=ORIENTED_EDGE('',*,*,#58103,.F.);
#85492=ORIENTED_EDGE('',*,*,#56213,.F.);
#85493=ORIENTED_EDGE('',*,*,#58102,.T.);
#85494=ORIENTED_EDGE('',*,*,#56232,.F.);
#85495=ORIENTED_EDGE('',*,*,#58104,.F.);
#85496=ORIENTED_EDGE('',*,*,#52871,.F.);
#85497=ORIENTED_EDGE('',*,*,#58103,.T.);
#85498=ORIENTED_EDGE('',*,*,#52404,.F.);
#85499=ORIENTED_EDGE('',*,*,#58105,.F.);
#85500=ORIENTED_EDGE('',*,*,#56522,.F.);
#85501=ORIENTED_EDGE('',*,*,#58104,.T.);
#85502=ORIENTED_EDGE('',*,*,#56231,.F.);
#85503=ORIENTED_EDGE('',*,*,#58106,.F.);
#85504=ORIENTED_EDGE('',*,*,#52620,.F.);
#85505=ORIENTED_EDGE('',*,*,#58105,.T.);
#85506=ORIENTED_EDGE('',*,*,#52403,.F.);
#85507=ORIENTED_EDGE('',*,*,#58107,.F.);
#85508=ORIENTED_EDGE('',*,*,#56219,.F.);
#85509=ORIENTED_EDGE('',*,*,#58106,.T.);
#85510=ORIENTED_EDGE('',*,*,#56521,.F.);
#85511=ORIENTED_EDGE('',*,*,#58108,.F.);
#85512=ORIENTED_EDGE('',*,*,#52621,.F.);
#85513=ORIENTED_EDGE('',*,*,#58107,.T.);
#85514=ORIENTED_EDGE('',*,*,#52902,.F.);
#85515=ORIENTED_EDGE('',*,*,#58109,.F.);
#85516=ORIENTED_EDGE('',*,*,#56220,.F.);
#85517=ORIENTED_EDGE('',*,*,#58108,.T.);
#85518=ORIENTED_EDGE('',*,*,#56215,.F.);
#85519=ORIENTED_EDGE('',*,*,#58110,.F.);
#85520=ORIENTED_EDGE('',*,*,#52622,.F.);
#85521=ORIENTED_EDGE('',*,*,#52897,.F.);
#85522=ORIENTED_EDGE('',*,*,#52893,.T.);
#85523=ORIENTED_EDGE('',*,*,#58111,.F.);
#85524=ORIENTED_EDGE('',*,*,#56221,.F.);
#85525=ORIENTED_EDGE('',*,*,#58109,.T.);
#85526=ORIENTED_EDGE('',*,*,#58110,.T.);
#85527=ORIENTED_EDGE('',*,*,#56523,.F.);
#85528=ORIENTED_EDGE('',*,*,#58112,.F.);
#85529=ORIENTED_EDGE('',*,*,#52623,.F.);
#85530=ORIENTED_EDGE('',*,*,#58111,.T.);
#85531=ORIENTED_EDGE('',*,*,#52892,.F.);
#85532=ORIENTED_EDGE('',*,*,#58113,.F.);
#85533=ORIENTED_EDGE('',*,*,#56222,.F.);
#85534=ORIENTED_EDGE('',*,*,#58112,.T.);
#85535=ORIENTED_EDGE('',*,*,#56217,.F.);
#85536=ORIENTED_EDGE('',*,*,#58114,.F.);
#85537=ORIENTED_EDGE('',*,*,#52624,.F.);
#85538=ORIENTED_EDGE('',*,*,#58113,.T.);
#85539=ORIENTED_EDGE('',*,*,#52904,.F.);
#85540=ORIENTED_EDGE('',*,*,#58115,.F.);
#85541=ORIENTED_EDGE('',*,*,#56223,.F.);
#85542=ORIENTED_EDGE('',*,*,#58114,.T.);
#85543=ORIENTED_EDGE('',*,*,#56216,.F.);
#85544=ORIENTED_EDGE('',*,*,#58116,.F.);
#85545=ORIENTED_EDGE('',*,*,#52900,.F.);
#85546=ORIENTED_EDGE('',*,*,#58115,.T.);
#85547=ORIENTED_EDGE('',*,*,#52888,.F.);
#85548=ORIENTED_EDGE('',*,*,#58117,.F.);
#85549=ORIENTED_EDGE('',*,*,#56224,.F.);
#85550=ORIENTED_EDGE('',*,*,#58116,.T.);
#85551=ORIENTED_EDGE('',*,*,#56227,.F.);
#85552=ORIENTED_EDGE('',*,*,#58118,.F.);
#85553=ORIENTED_EDGE('',*,*,#52879,.F.);
#85554=ORIENTED_EDGE('',*,*,#58117,.T.);
#85555=ORIENTED_EDGE('',*,*,#52906,.F.);
#85556=ORIENTED_EDGE('',*,*,#58119,.F.);
#85557=ORIENTED_EDGE('',*,*,#56225,.F.);
#85558=ORIENTED_EDGE('',*,*,#58118,.T.);
#85559=ORIENTED_EDGE('',*,*,#56226,.F.);
#85560=ORIENTED_EDGE('',*,*,#58119,.T.);
#85561=ORIENTED_EDGE('',*,*,#52884,.F.);
#85562=ORIENTED_EDGE('',*,*,#52880,.T.);
#85563=ORIENTED_EDGE('',*,*,#58120,.F.);
#85564=ORIENTED_EDGE('',*,*,#56266,.F.);
#85565=ORIENTED_EDGE('',*,*,#58121,.F.);
#85566=ORIENTED_EDGE('',*,*,#52836,.F.);
#85567=ORIENTED_EDGE('',*,*,#58121,.T.);
#85568=ORIENTED_EDGE('',*,*,#56265,.F.);
#85569=ORIENTED_EDGE('',*,*,#58122,.F.);
#85570=ORIENTED_EDGE('',*,*,#52845,.F.);
#85571=ORIENTED_EDGE('',*,*,#52835,.T.);
#85572=ORIENTED_EDGE('',*,*,#52839,.F.);
#85573=ORIENTED_EDGE('',*,*,#58123,.F.);
#85574=ORIENTED_EDGE('',*,*,#56267,.F.);
#85575=ORIENTED_EDGE('',*,*,#58120,.T.);
#85576=ORIENTED_EDGE('',*,*,#58122,.T.);
#85577=ORIENTED_EDGE('',*,*,#56264,.F.);
#85578=ORIENTED_EDGE('',*,*,#58124,.F.);
#85579=ORIENTED_EDGE('',*,*,#52830,.F.);
#85580=ORIENTED_EDGE('',*,*,#58123,.T.);
#85581=ORIENTED_EDGE('',*,*,#52843,.F.);
#85582=ORIENTED_EDGE('',*,*,#58125,.F.);
#85583=ORIENTED_EDGE('',*,*,#56256,.F.);
#85584=ORIENTED_EDGE('',*,*,#58124,.T.);
#85585=ORIENTED_EDGE('',*,*,#56263,.F.);
#85586=ORIENTED_EDGE('',*,*,#58126,.F.);
#85587=ORIENTED_EDGE('',*,*,#52847,.F.);
#85588=ORIENTED_EDGE('',*,*,#58125,.T.);
#85589=ORIENTED_EDGE('',*,*,#52413,.F.);
#85590=ORIENTED_EDGE('',*,*,#58127,.F.);
#85591=ORIENTED_EDGE('',*,*,#56257,.F.);
#85592=ORIENTED_EDGE('',*,*,#58126,.T.);
#85593=ORIENTED_EDGE('',*,*,#56262,.F.);
#85594=ORIENTED_EDGE('',*,*,#58128,.F.);
#85595=ORIENTED_EDGE('',*,*,#52822,.T.);
#85596=ORIENTED_EDGE('',*,*,#52826,.F.);
#85597=ORIENTED_EDGE('',*,*,#58127,.T.);
#85598=ORIENTED_EDGE('',*,*,#52412,.F.);
#85599=ORIENTED_EDGE('',*,*,#58129,.F.);
#85600=ORIENTED_EDGE('',*,*,#56524,.F.);
#85601=ORIENTED_EDGE('',*,*,#58128,.T.);
#85602=ORIENTED_EDGE('',*,*,#56261,.F.);
#85603=ORIENTED_EDGE('',*,*,#58130,.F.);
#85604=ORIENTED_EDGE('',*,*,#52823,.F.);
#85605=ORIENTED_EDGE('',*,*,#58129,.T.);
#85606=ORIENTED_EDGE('',*,*,#52411,.F.);
#85607=ORIENTED_EDGE('',*,*,#58131,.F.);
#85608=ORIENTED_EDGE('',*,*,#56241,.F.);
#85609=ORIENTED_EDGE('',*,*,#58130,.T.);
#85610=ORIENTED_EDGE('',*,*,#56260,.F.);
#85611=ORIENTED_EDGE('',*,*,#58132,.F.);
#85612=ORIENTED_EDGE('',*,*,#52841,.F.);
#85613=ORIENTED_EDGE('',*,*,#58131,.T.);
#85614=ORIENTED_EDGE('',*,*,#52410,.F.);
#85615=ORIENTED_EDGE('',*,*,#58133,.F.);
#85616=ORIENTED_EDGE('',*,*,#56526,.F.);
#85617=ORIENTED_EDGE('',*,*,#58132,.T.);
#85618=ORIENTED_EDGE('',*,*,#56259,.F.);
#85619=ORIENTED_EDGE('',*,*,#58134,.F.);
#85620=ORIENTED_EDGE('',*,*,#52614,.F.);
#85621=ORIENTED_EDGE('',*,*,#58133,.T.);
#85622=ORIENTED_EDGE('',*,*,#52409,.F.);
#85623=ORIENTED_EDGE('',*,*,#58135,.F.);
#85624=ORIENTED_EDGE('',*,*,#56247,.F.);
#85625=ORIENTED_EDGE('',*,*,#58134,.T.);
#85626=ORIENTED_EDGE('',*,*,#56525,.F.);
#85627=ORIENTED_EDGE('',*,*,#58136,.F.);
#85628=ORIENTED_EDGE('',*,*,#52615,.F.);
#85629=ORIENTED_EDGE('',*,*,#58135,.T.);
#85630=ORIENTED_EDGE('',*,*,#52872,.F.);
#85631=ORIENTED_EDGE('',*,*,#58137,.F.);
#85632=ORIENTED_EDGE('',*,*,#56248,.F.);
#85633=ORIENTED_EDGE('',*,*,#58136,.T.);
#85634=ORIENTED_EDGE('',*,*,#56243,.F.);
#85635=ORIENTED_EDGE('',*,*,#58138,.F.);
#85636=ORIENTED_EDGE('',*,*,#52616,.F.);
#85637=ORIENTED_EDGE('',*,*,#52867,.F.);
#85638=ORIENTED_EDGE('',*,*,#52863,.T.);
#85639=ORIENTED_EDGE('',*,*,#58139,.F.);
#85640=ORIENTED_EDGE('',*,*,#56249,.F.);
#85641=ORIENTED_EDGE('',*,*,#58137,.T.);
#85642=ORIENTED_EDGE('',*,*,#58138,.T.);
#85643=ORIENTED_EDGE('',*,*,#56527,.F.);
#85644=ORIENTED_EDGE('',*,*,#58140,.F.);
#85645=ORIENTED_EDGE('',*,*,#52617,.F.);
#85646=ORIENTED_EDGE('',*,*,#58139,.T.);
#85647=ORIENTED_EDGE('',*,*,#52862,.F.);
#85648=ORIENTED_EDGE('',*,*,#58141,.F.);
#85649=ORIENTED_EDGE('',*,*,#56250,.F.);
#85650=ORIENTED_EDGE('',*,*,#58140,.T.);
#85651=ORIENTED_EDGE('',*,*,#56245,.F.);
#85652=ORIENTED_EDGE('',*,*,#58142,.F.);
#85653=ORIENTED_EDGE('',*,*,#52618,.F.);
#85654=ORIENTED_EDGE('',*,*,#58141,.T.);
#85655=ORIENTED_EDGE('',*,*,#52874,.F.);
#85656=ORIENTED_EDGE('',*,*,#58143,.F.);
#85657=ORIENTED_EDGE('',*,*,#56251,.F.);
#85658=ORIENTED_EDGE('',*,*,#58142,.T.);
#85659=ORIENTED_EDGE('',*,*,#56244,.F.);
#85660=ORIENTED_EDGE('',*,*,#58144,.F.);
#85661=ORIENTED_EDGE('',*,*,#52870,.F.);
#85662=ORIENTED_EDGE('',*,*,#58143,.T.);
#85663=ORIENTED_EDGE('',*,*,#52858,.F.);
#85664=ORIENTED_EDGE('',*,*,#58145,.F.);
#85665=ORIENTED_EDGE('',*,*,#56252,.F.);
#85666=ORIENTED_EDGE('',*,*,#58144,.T.);
#85667=ORIENTED_EDGE('',*,*,#56255,.F.);
#85668=ORIENTED_EDGE('',*,*,#58146,.F.);
#85669=ORIENTED_EDGE('',*,*,#52849,.F.);
#85670=ORIENTED_EDGE('',*,*,#58145,.T.);
#85671=ORIENTED_EDGE('',*,*,#52876,.F.);
#85672=ORIENTED_EDGE('',*,*,#58147,.F.);
#85673=ORIENTED_EDGE('',*,*,#56253,.F.);
#85674=ORIENTED_EDGE('',*,*,#58146,.T.);
#85675=ORIENTED_EDGE('',*,*,#56254,.F.);
#85676=ORIENTED_EDGE('',*,*,#58147,.T.);
#85677=ORIENTED_EDGE('',*,*,#52854,.F.);
#85678=ORIENTED_EDGE('',*,*,#52850,.T.);
#85679=ORIENTED_EDGE('',*,*,#58148,.F.);
#85680=ORIENTED_EDGE('',*,*,#56294,.F.);
#85681=ORIENTED_EDGE('',*,*,#58149,.F.);
#85682=ORIENTED_EDGE('',*,*,#52802,.F.);
#85683=ORIENTED_EDGE('',*,*,#58149,.T.);
#85684=ORIENTED_EDGE('',*,*,#56293,.F.);
#85685=ORIENTED_EDGE('',*,*,#58150,.F.);
#85686=ORIENTED_EDGE('',*,*,#52814,.F.);
#85687=ORIENTED_EDGE('',*,*,#52801,.T.);
#85688=ORIENTED_EDGE('',*,*,#52808,.F.);
#85689=ORIENTED_EDGE('',*,*,#58151,.F.);
#85690=ORIENTED_EDGE('',*,*,#56295,.F.);
#85691=ORIENTED_EDGE('',*,*,#58148,.T.);
#85692=ORIENTED_EDGE('',*,*,#58150,.T.);
#85693=ORIENTED_EDGE('',*,*,#56292,.F.);
#85694=ORIENTED_EDGE('',*,*,#58152,.F.);
#85695=ORIENTED_EDGE('',*,*,#52798,.F.);
#85696=ORIENTED_EDGE('',*,*,#58151,.T.);
#85697=ORIENTED_EDGE('',*,*,#52812,.F.);
#85698=ORIENTED_EDGE('',*,*,#58153,.F.);
#85699=ORIENTED_EDGE('',*,*,#56284,.F.);
#85700=ORIENTED_EDGE('',*,*,#58152,.T.);
#85701=ORIENTED_EDGE('',*,*,#56291,.F.);
#85702=ORIENTED_EDGE('',*,*,#58154,.F.);
#85703=ORIENTED_EDGE('',*,*,#52816,.F.);
#85704=ORIENTED_EDGE('',*,*,#58153,.T.);
#85705=ORIENTED_EDGE('',*,*,#52419,.F.);
#85706=ORIENTED_EDGE('',*,*,#58155,.F.);
#85707=ORIENTED_EDGE('',*,*,#56285,.F.);
#85708=ORIENTED_EDGE('',*,*,#58154,.T.);
#85709=ORIENTED_EDGE('',*,*,#56290,.F.);
#85710=ORIENTED_EDGE('',*,*,#58156,.F.);
#85711=ORIENTED_EDGE('',*,*,#52788,.T.);
#85712=ORIENTED_EDGE('',*,*,#52795,.F.);
#85713=ORIENTED_EDGE('',*,*,#58155,.T.);
#85714=ORIENTED_EDGE('',*,*,#52418,.F.);
#85715=ORIENTED_EDGE('',*,*,#58157,.F.);
#85716=ORIENTED_EDGE('',*,*,#56528,.F.);
#85717=ORIENTED_EDGE('',*,*,#58156,.T.);
#85718=ORIENTED_EDGE('',*,*,#56289,.F.);
#85719=ORIENTED_EDGE('',*,*,#58158,.F.);
#85720=ORIENTED_EDGE('',*,*,#52789,.F.);
#85721=ORIENTED_EDGE('',*,*,#58157,.T.);
#85722=ORIENTED_EDGE('',*,*,#52417,.F.);
#85723=ORIENTED_EDGE('',*,*,#58159,.F.);
#85724=ORIENTED_EDGE('',*,*,#56269,.F.);
#85725=ORIENTED_EDGE('',*,*,#58158,.T.);
#85726=ORIENTED_EDGE('',*,*,#56288,.F.);
#85727=ORIENTED_EDGE('',*,*,#58160,.F.);
#85728=ORIENTED_EDGE('',*,*,#52810,.F.);
#85729=ORIENTED_EDGE('',*,*,#58159,.T.);
#85730=ORIENTED_EDGE('',*,*,#52416,.F.);
#85731=ORIENTED_EDGE('',*,*,#58161,.F.);
#85732=ORIENTED_EDGE('',*,*,#56530,.F.);
#85733=ORIENTED_EDGE('',*,*,#58160,.T.);
#85734=ORIENTED_EDGE('',*,*,#56287,.F.);
#85735=ORIENTED_EDGE('',*,*,#58162,.F.);
#85736=ORIENTED_EDGE('',*,*,#52608,.F.);
#85737=ORIENTED_EDGE('',*,*,#58161,.T.);
#85738=ORIENTED_EDGE('',*,*,#52415,.F.);
#85739=ORIENTED_EDGE('',*,*,#58163,.F.);
#85740=ORIENTED_EDGE('',*,*,#56275,.F.);
#85741=ORIENTED_EDGE('',*,*,#58162,.T.);
#85742=ORIENTED_EDGE('',*,*,#56529,.F.);
#85743=ORIENTED_EDGE('',*,*,#58164,.F.);
#85744=ORIENTED_EDGE('',*,*,#52609,.F.);
#85745=ORIENTED_EDGE('',*,*,#58163,.T.);
#85746=ORIENTED_EDGE('',*,*,#52842,.F.);
#85747=ORIENTED_EDGE('',*,*,#58165,.F.);
#85748=ORIENTED_EDGE('',*,*,#56276,.F.);
#85749=ORIENTED_EDGE('',*,*,#58164,.T.);
#85750=ORIENTED_EDGE('',*,*,#56271,.F.);
#85751=ORIENTED_EDGE('',*,*,#58166,.F.);
#85752=ORIENTED_EDGE('',*,*,#52610,.F.);
#85753=ORIENTED_EDGE('',*,*,#52837,.F.);
#85754=ORIENTED_EDGE('',*,*,#52833,.T.);
#85755=ORIENTED_EDGE('',*,*,#58167,.F.);
#85756=ORIENTED_EDGE('',*,*,#56277,.F.);
#85757=ORIENTED_EDGE('',*,*,#58165,.T.);
#85758=ORIENTED_EDGE('',*,*,#58166,.T.);
#85759=ORIENTED_EDGE('',*,*,#56531,.F.);
#85760=ORIENTED_EDGE('',*,*,#58168,.F.);
#85761=ORIENTED_EDGE('',*,*,#52611,.F.);
#85762=ORIENTED_EDGE('',*,*,#58167,.T.);
#85763=ORIENTED_EDGE('',*,*,#52832,.F.);
#85764=ORIENTED_EDGE('',*,*,#58169,.F.);
#85765=ORIENTED_EDGE('',*,*,#56278,.F.);
#85766=ORIENTED_EDGE('',*,*,#58168,.T.);
#85767=ORIENTED_EDGE('',*,*,#56273,.F.);
#85768=ORIENTED_EDGE('',*,*,#58170,.F.);
#85769=ORIENTED_EDGE('',*,*,#52612,.F.);
#85770=ORIENTED_EDGE('',*,*,#58169,.T.);
#85771=ORIENTED_EDGE('',*,*,#52844,.F.);
#85772=ORIENTED_EDGE('',*,*,#58171,.F.);
#85773=ORIENTED_EDGE('',*,*,#56279,.F.);
#85774=ORIENTED_EDGE('',*,*,#58170,.T.);
#85775=ORIENTED_EDGE('',*,*,#56272,.F.);
#85776=ORIENTED_EDGE('',*,*,#58172,.F.);
#85777=ORIENTED_EDGE('',*,*,#52840,.F.);
#85778=ORIENTED_EDGE('',*,*,#58171,.T.);
#85779=ORIENTED_EDGE('',*,*,#52828,.F.);
#85780=ORIENTED_EDGE('',*,*,#58173,.F.);
#85781=ORIENTED_EDGE('',*,*,#56280,.F.);
#85782=ORIENTED_EDGE('',*,*,#58172,.T.);
#85783=ORIENTED_EDGE('',*,*,#56283,.F.);
#85784=ORIENTED_EDGE('',*,*,#58174,.F.);
#85785=ORIENTED_EDGE('',*,*,#52819,.F.);
#85786=ORIENTED_EDGE('',*,*,#58173,.T.);
#85787=ORIENTED_EDGE('',*,*,#52846,.F.);
#85788=ORIENTED_EDGE('',*,*,#58175,.F.);
#85789=ORIENTED_EDGE('',*,*,#56281,.F.);
#85790=ORIENTED_EDGE('',*,*,#58174,.T.);
#85791=ORIENTED_EDGE('',*,*,#56282,.F.);
#85792=ORIENTED_EDGE('',*,*,#58175,.T.);
#85793=ORIENTED_EDGE('',*,*,#52824,.F.);
#85794=ORIENTED_EDGE('',*,*,#52820,.T.);
#85795=ORIENTED_EDGE('',*,*,#58176,.F.);
#85796=ORIENTED_EDGE('',*,*,#58177,.T.);
#85797=ORIENTED_EDGE('',*,*,#58178,.F.);
#85798=ORIENTED_EDGE('',*,*,#58177,.F.);
#85799=ORIENTED_EDGE('',*,*,#58179,.F.);
#85800=ORIENTED_EDGE('',*,*,#58180,.T.);
#85801=ORIENTED_EDGE('',*,*,#58181,.F.);
#85802=ORIENTED_EDGE('',*,*,#58180,.F.);
#85803=ORIENTED_EDGE('',*,*,#58182,.F.);
#85804=ORIENTED_EDGE('',*,*,#58183,.T.);
#85805=ORIENTED_EDGE('',*,*,#58184,.F.);
#85806=ORIENTED_EDGE('',*,*,#58185,.F.);
#85807=ORIENTED_EDGE('',*,*,#58183,.F.);
#85808=ORIENTED_EDGE('',*,*,#58186,.F.);
#85809=ORIENTED_EDGE('',*,*,#58187,.T.);
#85810=ORIENTED_EDGE('',*,*,#58176,.T.);
#85811=ORIENTED_EDGE('',*,*,#58187,.F.);
#85812=ORIENTED_EDGE('',*,*,#58181,.T.);
#85813=ORIENTED_EDGE('',*,*,#58188,.T.);
#85814=ORIENTED_EDGE('',*,*,#58184,.T.);
#85815=ORIENTED_EDGE('',*,*,#58185,.T.);
#85816=ORIENTED_EDGE('',*,*,#58188,.F.);
#85817=ORIENTED_EDGE('',*,*,#58189,.T.);
#85818=ORIENTED_EDGE('',*,*,#58190,.T.);
#85819=ORIENTED_EDGE('',*,*,#58191,.F.);
#85820=ORIENTED_EDGE('',*,*,#58190,.F.);
#85821=ORIENTED_EDGE('',*,*,#58191,.T.);
#85822=ORIENTED_EDGE('',*,*,#58186,.T.);
#85823=ORIENTED_EDGE('',*,*,#58189,.F.);
#85824=ORIENTED_EDGE('',*,*,#58182,.T.);
#85825=ORIENTED_EDGE('',*,*,#58179,.T.);
#85826=ORIENTED_EDGE('',*,*,#58178,.T.);
#85827=ORIENTED_EDGE('',*,*,#58192,.F.);
#85828=ORIENTED_EDGE('',*,*,#58193,.T.);
#85829=ORIENTED_EDGE('',*,*,#58194,.F.);
#85830=ORIENTED_EDGE('',*,*,#58193,.F.);
#85831=ORIENTED_EDGE('',*,*,#58195,.F.);
#85832=ORIENTED_EDGE('',*,*,#58196,.T.);
#85833=ORIENTED_EDGE('',*,*,#58197,.F.);
#85834=ORIENTED_EDGE('',*,*,#58196,.F.);
#85835=ORIENTED_EDGE('',*,*,#58198,.F.);
#85836=ORIENTED_EDGE('',*,*,#58199,.T.);
#85837=ORIENTED_EDGE('',*,*,#58192,.T.);
#85838=ORIENTED_EDGE('',*,*,#58199,.F.);
#85839=ORIENTED_EDGE('',*,*,#58197,.T.);
#85840=ORIENTED_EDGE('',*,*,#58200,.T.);
#85841=ORIENTED_EDGE('',*,*,#58201,.T.);
#85842=ORIENTED_EDGE('',*,*,#58200,.F.);
#85843=ORIENTED_EDGE('',*,*,#58201,.F.);
#85844=ORIENTED_EDGE('',*,*,#58198,.T.);
#85845=ORIENTED_EDGE('',*,*,#58195,.T.);
#85846=ORIENTED_EDGE('',*,*,#58194,.T.);
#85847=ORIENTED_EDGE('',*,*,#58202,.T.);
#85848=ORIENTED_EDGE('',*,*,#58203,.T.);
#85849=ORIENTED_EDGE('',*,*,#58204,.F.);
#85850=ORIENTED_EDGE('',*,*,#58203,.F.);
#85851=ORIENTED_EDGE('',*,*,#58205,.F.);
#85852=ORIENTED_EDGE('',*,*,#58206,.F.);
#85853=ORIENTED_EDGE('',*,*,#58207,.F.);
#85854=ORIENTED_EDGE('',*,*,#58208,.T.);
#85855=ORIENTED_EDGE('',*,*,#58209,.F.);
#85856=ORIENTED_EDGE('',*,*,#58210,.T.);
#85857=ORIENTED_EDGE('',*,*,#58211,.F.);
#85858=ORIENTED_EDGE('',*,*,#58212,.F.);
#85859=ORIENTED_EDGE('',*,*,#58213,.F.);
#85860=ORIENTED_EDGE('',*,*,#58214,.T.);
#85861=ORIENTED_EDGE('',*,*,#58215,.F.);
#85862=ORIENTED_EDGE('',*,*,#58216,.F.);
#85863=ORIENTED_EDGE('',*,*,#58217,.F.);
#85864=ORIENTED_EDGE('',*,*,#58218,.T.);
#85865=ORIENTED_EDGE('',*,*,#58219,.F.);
#85866=ORIENTED_EDGE('',*,*,#58220,.F.);
#85867=ORIENTED_EDGE('',*,*,#58221,.F.);
#85868=ORIENTED_EDGE('',*,*,#58222,.F.);
#85869=ORIENTED_EDGE('',*,*,#58223,.F.);
#85870=ORIENTED_EDGE('',*,*,#58224,.F.);
#85871=ORIENTED_EDGE('',*,*,#58225,.F.);
#85872=ORIENTED_EDGE('',*,*,#58226,.T.);
#85873=ORIENTED_EDGE('',*,*,#58227,.F.);
#85874=ORIENTED_EDGE('',*,*,#58228,.F.);
#85875=ORIENTED_EDGE('',*,*,#58229,.F.);
#85876=ORIENTED_EDGE('',*,*,#58226,.F.);
#85877=ORIENTED_EDGE('',*,*,#58230,.F.);
#85878=ORIENTED_EDGE('',*,*,#58231,.T.);
#85879=ORIENTED_EDGE('',*,*,#58232,.F.);
#85880=ORIENTED_EDGE('',*,*,#58233,.F.);
#85881=ORIENTED_EDGE('',*,*,#58234,.F.);
#85882=ORIENTED_EDGE('',*,*,#58231,.F.);
#85883=ORIENTED_EDGE('',*,*,#58219,.T.);
#85884=ORIENTED_EDGE('',*,*,#58235,.F.);
#85885=ORIENTED_EDGE('',*,*,#58236,.F.);
#85886=ORIENTED_EDGE('',*,*,#58237,.T.);
#85887=ORIENTED_EDGE('',*,*,#58238,.T.);
#85888=ORIENTED_EDGE('',*,*,#58239,.F.);
#85889=ORIENTED_EDGE('',*,*,#58223,.T.);
#85890=ORIENTED_EDGE('',*,*,#58240,.F.);
#85891=ORIENTED_EDGE('',*,*,#58241,.T.);
#85892=ORIENTED_EDGE('',*,*,#58242,.T.);
#85893=ORIENTED_EDGE('',*,*,#58243,.F.);
#85894=ORIENTED_EDGE('',*,*,#58244,.F.);
#85895=ORIENTED_EDGE('',*,*,#58245,.F.);
#85896=ORIENTED_EDGE('',*,*,#58246,.T.);
#85897=ORIENTED_EDGE('',*,*,#58247,.F.);
#85898=ORIENTED_EDGE('',*,*,#58248,.T.);
#85899=ORIENTED_EDGE('',*,*,#58249,.F.);
#85900=ORIENTED_EDGE('',*,*,#58250,.T.);
#85901=ORIENTED_EDGE('',*,*,#58251,.T.);
#85902=ORIENTED_EDGE('',*,*,#58250,.F.);
#85903=ORIENTED_EDGE('',*,*,#58252,.T.);
#85904=ORIENTED_EDGE('',*,*,#58253,.T.);
#85905=ORIENTED_EDGE('',*,*,#58254,.T.);
#85906=ORIENTED_EDGE('',*,*,#58253,.F.);
#85907=ORIENTED_EDGE('',*,*,#58255,.T.);
#85908=ORIENTED_EDGE('',*,*,#58256,.T.);
#85909=ORIENTED_EDGE('',*,*,#58257,.T.);
#85910=ORIENTED_EDGE('',*,*,#58256,.F.);
#85911=ORIENTED_EDGE('',*,*,#58258,.T.);
#85912=ORIENTED_EDGE('',*,*,#58259,.T.);
#85913=ORIENTED_EDGE('',*,*,#58260,.T.);
#85914=ORIENTED_EDGE('',*,*,#58259,.F.);
#85915=ORIENTED_EDGE('',*,*,#58261,.T.);
#85916=ORIENTED_EDGE('',*,*,#58262,.T.);
#85917=ORIENTED_EDGE('',*,*,#58263,.T.);
#85918=ORIENTED_EDGE('',*,*,#58262,.F.);
#85919=ORIENTED_EDGE('',*,*,#58229,.T.);
#85920=ORIENTED_EDGE('',*,*,#58264,.T.);
#85921=ORIENTED_EDGE('',*,*,#58265,.T.);
#85922=ORIENTED_EDGE('',*,*,#58266,.T.);
#85923=ORIENTED_EDGE('',*,*,#58205,.T.);
#85924=ORIENTED_EDGE('',*,*,#58267,.T.);
#85925=ORIENTED_EDGE('',*,*,#58268,.T.);
#85926=ORIENTED_EDGE('',*,*,#58269,.T.);
#85927=ORIENTED_EDGE('',*,*,#58270,.T.);
#85928=ORIENTED_EDGE('',*,*,#58271,.T.);
#85929=ORIENTED_EDGE('',*,*,#58272,.T.);
#85930=ORIENTED_EDGE('',*,*,#58273,.T.);
#85931=ORIENTED_EDGE('',*,*,#58245,.T.);
#85932=ORIENTED_EDGE('',*,*,#58274,.T.);
#85933=ORIENTED_EDGE('',*,*,#58275,.T.);
#85934=ORIENTED_EDGE('',*,*,#58276,.T.);
#85935=ORIENTED_EDGE('',*,*,#58277,.T.);
#85936=ORIENTED_EDGE('',*,*,#58278,.T.);
#85937=ORIENTED_EDGE('',*,*,#58279,.T.);
#85938=ORIENTED_EDGE('',*,*,#58280,.T.);
#85939=ORIENTED_EDGE('',*,*,#58281,.T.);
#85940=ORIENTED_EDGE('',*,*,#58282,.T.);
#85941=ORIENTED_EDGE('',*,*,#58283,.T.);
#85942=ORIENTED_EDGE('',*,*,#58284,.T.);
#85943=ORIENTED_EDGE('',*,*,#58285,.T.);
#85944=ORIENTED_EDGE('',*,*,#58286,.T.);
#85945=ORIENTED_EDGE('',*,*,#58287,.T.);
#85946=ORIENTED_EDGE('',*,*,#58288,.T.);
#85947=ORIENTED_EDGE('',*,*,#58289,.T.);
#85948=ORIENTED_EDGE('',*,*,#58290,.T.);
#85949=ORIENTED_EDGE('',*,*,#58291,.T.);
#85950=ORIENTED_EDGE('',*,*,#58292,.T.);
#85951=ORIENTED_EDGE('',*,*,#58293,.T.);
#85952=ORIENTED_EDGE('',*,*,#58294,.F.);
#85953=ORIENTED_EDGE('',*,*,#58295,.T.);
#85954=ORIENTED_EDGE('',*,*,#58296,.T.);
#85955=ORIENTED_EDGE('',*,*,#58297,.T.);
#85956=ORIENTED_EDGE('',*,*,#58298,.F.);
#85957=ORIENTED_EDGE('',*,*,#58299,.F.);
#85958=ORIENTED_EDGE('',*,*,#58300,.T.);
#85959=ORIENTED_EDGE('',*,*,#58301,.T.);
#85960=ORIENTED_EDGE('',*,*,#58302,.T.);
#85961=ORIENTED_EDGE('',*,*,#58303,.T.);
#85962=ORIENTED_EDGE('',*,*,#58304,.F.);
#85963=ORIENTED_EDGE('',*,*,#58305,.T.);
#85964=ORIENTED_EDGE('',*,*,#58306,.T.);
#85965=ORIENTED_EDGE('',*,*,#58307,.T.);
#85966=ORIENTED_EDGE('',*,*,#58308,.F.);
#85967=ORIENTED_EDGE('',*,*,#58309,.F.);
#85968=ORIENTED_EDGE('',*,*,#58310,.T.);
#85969=ORIENTED_EDGE('',*,*,#58311,.T.);
#85970=ORIENTED_EDGE('',*,*,#58312,.T.);
#85971=ORIENTED_EDGE('',*,*,#58313,.F.);
#85972=ORIENTED_EDGE('',*,*,#58314,.T.);
#85973=ORIENTED_EDGE('',*,*,#58309,.T.);
#85974=ORIENTED_EDGE('',*,*,#58315,.F.);
#85975=ORIENTED_EDGE('',*,*,#58307,.F.);
#85976=ORIENTED_EDGE('',*,*,#58316,.T.);
#85977=ORIENTED_EDGE('',*,*,#58299,.T.);
#85978=ORIENTED_EDGE('',*,*,#58317,.F.);
#85979=ORIENTED_EDGE('',*,*,#58318,.F.);
#85980=ORIENTED_EDGE('',*,*,#58319,.T.);
#85981=ORIENTED_EDGE('',*,*,#58320,.T.);
#85982=ORIENTED_EDGE('',*,*,#58321,.F.);
#85983=ORIENTED_EDGE('',*,*,#58322,.T.);
#85984=ORIENTED_EDGE('',*,*,#58209,.T.);
#85985=ORIENTED_EDGE('',*,*,#58323,.F.);
#85986=ORIENTED_EDGE('',*,*,#58324,.T.);
#85987=ORIENTED_EDGE('',*,*,#58325,.T.);
#85988=ORIENTED_EDGE('',*,*,#58313,.T.);
#85989=ORIENTED_EDGE('',*,*,#58326,.F.);
#85990=ORIENTED_EDGE('',*,*,#58320,.F.);
#85991=ORIENTED_EDGE('',*,*,#58327,.T.);
#85992=ORIENTED_EDGE('',*,*,#58328,.T.);
#85993=ORIENTED_EDGE('',*,*,#58329,.T.);
#85994=ORIENTED_EDGE('',*,*,#58213,.T.);
#85995=ORIENTED_EDGE('',*,*,#58330,.F.);
#85996=ORIENTED_EDGE('',*,*,#58331,.T.);
#85997=ORIENTED_EDGE('',*,*,#58332,.T.);
#85998=ORIENTED_EDGE('',*,*,#58318,.T.);
#85999=ORIENTED_EDGE('',*,*,#58333,.F.);
#86000=ORIENTED_EDGE('',*,*,#58334,.F.);
#86001=ORIENTED_EDGE('',*,*,#58335,.T.);
#86002=ORIENTED_EDGE('',*,*,#58336,.T.);
#86003=ORIENTED_EDGE('',*,*,#58337,.T.);
#86004=ORIENTED_EDGE('',*,*,#58338,.T.);
#86005=ORIENTED_EDGE('',*,*,#58334,.T.);
#86006=ORIENTED_EDGE('',*,*,#58339,.F.);
#86007=ORIENTED_EDGE('',*,*,#58297,.F.);
#86008=ORIENTED_EDGE('',*,*,#58340,.T.);
#86009=ORIENTED_EDGE('',*,*,#58341,.F.);
#86010=ORIENTED_EDGE('',*,*,#58342,.T.);
#86011=ORIENTED_EDGE('',*,*,#58343,.T.);
#86012=ORIENTED_EDGE('',*,*,#58344,.F.);
#86013=ORIENTED_EDGE('',*,*,#58343,.F.);
#86014=ORIENTED_EDGE('',*,*,#58345,.T.);
#86015=ORIENTED_EDGE('',*,*,#58346,.T.);
#86016=ORIENTED_EDGE('',*,*,#58347,.F.);
#86017=ORIENTED_EDGE('',*,*,#58346,.F.);
#86018=ORIENTED_EDGE('',*,*,#58348,.T.);
#86019=ORIENTED_EDGE('',*,*,#58349,.T.);
#86020=ORIENTED_EDGE('',*,*,#58350,.F.);
#86021=ORIENTED_EDGE('',*,*,#58349,.F.);
#86022=ORIENTED_EDGE('',*,*,#58351,.T.);
#86023=ORIENTED_EDGE('',*,*,#58352,.T.);
#86024=ORIENTED_EDGE('',*,*,#58353,.F.);
#86025=ORIENTED_EDGE('',*,*,#58352,.F.);
#86026=ORIENTED_EDGE('',*,*,#58354,.T.);
#86027=ORIENTED_EDGE('',*,*,#58355,.T.);
#86028=ORIENTED_EDGE('',*,*,#58356,.F.);
#86029=ORIENTED_EDGE('',*,*,#58355,.F.);
#86030=ORIENTED_EDGE('',*,*,#58357,.T.);
#86031=ORIENTED_EDGE('',*,*,#58358,.T.);
#86032=ORIENTED_EDGE('',*,*,#58359,.F.);
#86033=ORIENTED_EDGE('',*,*,#58358,.F.);
#86034=ORIENTED_EDGE('',*,*,#58360,.T.);
#86035=ORIENTED_EDGE('',*,*,#58361,.T.);
#86036=ORIENTED_EDGE('',*,*,#58362,.F.);
#86037=ORIENTED_EDGE('',*,*,#58361,.F.);
#86038=ORIENTED_EDGE('',*,*,#58363,.T.);
#86039=ORIENTED_EDGE('',*,*,#58341,.T.);
#86040=ORIENTED_EDGE('',*,*,#58364,.F.);
#86041=ORIENTED_EDGE('',*,*,#58365,.T.);
#86042=ORIENTED_EDGE('',*,*,#58366,.T.);
#86043=ORIENTED_EDGE('',*,*,#58367,.T.);
#86044=ORIENTED_EDGE('',*,*,#58368,.T.);
#86045=ORIENTED_EDGE('',*,*,#58369,.T.);
#86046=ORIENTED_EDGE('',*,*,#58207,.T.);
#86047=ORIENTED_EDGE('',*,*,#58204,.T.);
#86048=ORIENTED_EDGE('',*,*,#58370,.T.);
#86049=ORIENTED_EDGE('',*,*,#58371,.T.);
#86050=ORIENTED_EDGE('',*,*,#58372,.F.);
#86051=ORIENTED_EDGE('',*,*,#58373,.T.);
#86052=ORIENTED_EDGE('',*,*,#58374,.T.);
#86053=ORIENTED_EDGE('',*,*,#58375,.T.);
#86054=ORIENTED_EDGE('',*,*,#58376,.T.);
#86055=ORIENTED_EDGE('',*,*,#58377,.T.);
#86056=ORIENTED_EDGE('',*,*,#58378,.T.);
#86057=ORIENTED_EDGE('',*,*,#58379,.T.);
#86058=ORIENTED_EDGE('',*,*,#58380,.T.);
#86059=ORIENTED_EDGE('',*,*,#58381,.T.);
#86060=ORIENTED_EDGE('',*,*,#58382,.T.);
#86061=ORIENTED_EDGE('',*,*,#58383,.T.);
#86062=ORIENTED_EDGE('',*,*,#58384,.T.);
#86063=ORIENTED_EDGE('',*,*,#58385,.T.);
#86064=ORIENTED_EDGE('',*,*,#58372,.T.);
#86065=ORIENTED_EDGE('',*,*,#58386,.T.);
#86066=ORIENTED_EDGE('',*,*,#58378,.F.);
#86067=ORIENTED_EDGE('',*,*,#58387,.T.);
#86068=ORIENTED_EDGE('',*,*,#58374,.F.);
#86069=ORIENTED_EDGE('',*,*,#58388,.T.);
#86070=ORIENTED_EDGE('',*,*,#58384,.F.);
#86071=ORIENTED_EDGE('',*,*,#58389,.T.);
#86072=ORIENTED_EDGE('',*,*,#58390,.T.);
#86073=ORIENTED_EDGE('',*,*,#58391,.T.);
#86074=ORIENTED_EDGE('',*,*,#58392,.T.);
#86075=ORIENTED_EDGE('',*,*,#58393,.T.);
#86076=ORIENTED_EDGE('',*,*,#58394,.T.);
#86077=ORIENTED_EDGE('',*,*,#58395,.T.);
#86078=ORIENTED_EDGE('',*,*,#58396,.T.);
#86079=ORIENTED_EDGE('',*,*,#58397,.T.);
#86080=ORIENTED_EDGE('',*,*,#58398,.T.);
#86081=ORIENTED_EDGE('',*,*,#58392,.F.);
#86082=ORIENTED_EDGE('',*,*,#58399,.T.);
#86083=ORIENTED_EDGE('',*,*,#58400,.F.);
#86084=ORIENTED_EDGE('',*,*,#58336,.F.);
#86085=ORIENTED_EDGE('',*,*,#58401,.T.);
#86086=ORIENTED_EDGE('',*,*,#58402,.T.);
#86087=ORIENTED_EDGE('',*,*,#58403,.T.);
#86088=ORIENTED_EDGE('',*,*,#58295,.F.);
#86089=ORIENTED_EDGE('',*,*,#58404,.F.);
#86090=ORIENTED_EDGE('',*,*,#58405,.T.);
#86091=ORIENTED_EDGE('',*,*,#58406,.F.);
#86092=ORIENTED_EDGE('',*,*,#58407,.T.);
#86093=ORIENTED_EDGE('',*,*,#58408,.T.);
#86094=ORIENTED_EDGE('',*,*,#58406,.T.);
#86095=ORIENTED_EDGE('',*,*,#58409,.T.);
#86096=ORIENTED_EDGE('',*,*,#58410,.T.);
#86097=ORIENTED_EDGE('',*,*,#58411,.T.);
#86098=ORIENTED_EDGE('',*,*,#58412,.T.);
#86099=ORIENTED_EDGE('',*,*,#58413,.T.);
#86100=ORIENTED_EDGE('',*,*,#58255,.F.);
#86101=ORIENTED_EDGE('',*,*,#58235,.T.);
#86102=ORIENTED_EDGE('',*,*,#58414,.T.);
#86103=ORIENTED_EDGE('',*,*,#58244,.T.);
#86104=ORIENTED_EDGE('',*,*,#58247,.T.);
#86105=ORIENTED_EDGE('',*,*,#58415,.T.);
#86106=ORIENTED_EDGE('',*,*,#58416,.T.);
#86107=ORIENTED_EDGE('',*,*,#58417,.T.);
#86108=ORIENTED_EDGE('',*,*,#58418,.T.);
#86109=ORIENTED_EDGE('',*,*,#58252,.F.);
#86110=ORIENTED_EDGE('',*,*,#58419,.T.);
#86111=ORIENTED_EDGE('',*,*,#58420,.T.);
#86112=ORIENTED_EDGE('',*,*,#58421,.T.);
#86113=ORIENTED_EDGE('',*,*,#58422,.T.);
#86114=ORIENTED_EDGE('',*,*,#58423,.T.);
#86115=ORIENTED_EDGE('',*,*,#58424,.T.);
#86116=ORIENTED_EDGE('',*,*,#58425,.T.);
#86117=ORIENTED_EDGE('',*,*,#58211,.T.);
#86118=ORIENTED_EDGE('',*,*,#58261,.F.);
#86119=ORIENTED_EDGE('',*,*,#58426,.T.);
#86120=ORIENTED_EDGE('',*,*,#58427,.T.);
#86121=ORIENTED_EDGE('',*,*,#58428,.T.);
#86122=ORIENTED_EDGE('',*,*,#58215,.T.);
#86123=ORIENTED_EDGE('',*,*,#58258,.F.);
#86124=ORIENTED_EDGE('',*,*,#58429,.T.);
#86125=ORIENTED_EDGE('',*,*,#58430,.T.);
#86126=ORIENTED_EDGE('',*,*,#58431,.T.);
#86127=ORIENTED_EDGE('',*,*,#58432,.T.);
#86128=ORIENTED_EDGE('',*,*,#58329,.F.);
#86129=ORIENTED_EDGE('',*,*,#58400,.T.);
#86130=ORIENTED_EDGE('',*,*,#58433,.T.);
#86131=ORIENTED_EDGE('',*,*,#58434,.T.);
#86132=ORIENTED_EDGE('',*,*,#58435,.T.);
#86133=ORIENTED_EDGE('',*,*,#58436,.T.);
#86134=ORIENTED_EDGE('',*,*,#58404,.T.);
#86135=ORIENTED_EDGE('',*,*,#58294,.T.);
#86136=ORIENTED_EDGE('',*,*,#58239,.T.);
#86137=ORIENTED_EDGE('',*,*,#58437,.T.);
#86138=ORIENTED_EDGE('',*,*,#58438,.T.);
#86139=ORIENTED_EDGE('',*,*,#58439,.T.);
#86140=ORIENTED_EDGE('',*,*,#58302,.F.);
#86141=ORIENTED_EDGE('',*,*,#58440,.T.);
#86142=ORIENTED_EDGE('',*,*,#58441,.T.);
#86143=ORIENTED_EDGE('',*,*,#58442,.T.);
#86144=ORIENTED_EDGE('',*,*,#58443,.T.);
#86145=ORIENTED_EDGE('',*,*,#58444,.T.);
#86146=ORIENTED_EDGE('',*,*,#58221,.T.);
#86147=ORIENTED_EDGE('',*,*,#58445,.T.);
#86148=ORIENTED_EDGE('',*,*,#58217,.T.);
#86149=ORIENTED_EDGE('',*,*,#58446,.T.);
#86150=ORIENTED_EDGE('',*,*,#58447,.T.);
#86151=ORIENTED_EDGE('',*,*,#58448,.T.);
#86152=ORIENTED_EDGE('',*,*,#58449,.T.);
#86153=ORIENTED_EDGE('',*,*,#58240,.T.);
#86154=ORIENTED_EDGE('',*,*,#58450,.T.);
#86155=ORIENTED_EDGE('',*,*,#58304,.T.);
#86156=ORIENTED_EDGE('',*,*,#58451,.T.);
#86157=ORIENTED_EDGE('',*,*,#58452,.T.);
#86158=ORIENTED_EDGE('',*,*,#58453,.T.);
#86159=ORIENTED_EDGE('',*,*,#58454,.T.);
#86160=ORIENTED_EDGE('',*,*,#58312,.F.);
#86161=ORIENTED_EDGE('',*,*,#58455,.T.);
#86162=ORIENTED_EDGE('',*,*,#58456,.T.);
#86163=ORIENTED_EDGE('',*,*,#58457,.T.);
#86164=ORIENTED_EDGE('',*,*,#58458,.T.);
#86165=ORIENTED_EDGE('',*,*,#58459,.T.);
#86166=ORIENTED_EDGE('',*,*,#58460,.T.);
#86167=ORIENTED_EDGE('',*,*,#58461,.T.);
#86168=ORIENTED_EDGE('',*,*,#58462,.T.);
#86169=ORIENTED_EDGE('',*,*,#58463,.T.);
#86170=ORIENTED_EDGE('',*,*,#58464,.T.);
#86171=ORIENTED_EDGE('',*,*,#58465,.T.);
#86172=ORIENTED_EDGE('',*,*,#58466,.T.);
#86173=ORIENTED_EDGE('',*,*,#58467,.T.);
#86174=ORIENTED_EDGE('',*,*,#58468,.T.);
#86175=ORIENTED_EDGE('',*,*,#58323,.T.);
#86176=ORIENTED_EDGE('',*,*,#58469,.T.);
#86177=ORIENTED_EDGE('',*,*,#58470,.T.);
#86178=ORIENTED_EDGE('',*,*,#58471,.T.);
#86179=ORIENTED_EDGE('',*,*,#58472,.T.);
#86180=ORIENTED_EDGE('',*,*,#58322,.F.);
#86181=ORIENTED_EDGE('',*,*,#58473,.T.);
#86182=ORIENTED_EDGE('',*,*,#58474,.T.);
#86183=ORIENTED_EDGE('',*,*,#58475,.T.);
#86184=ORIENTED_EDGE('',*,*,#58476,.T.);
#86185=ORIENTED_EDGE('',*,*,#58477,.T.);
#86186=ORIENTED_EDGE('',*,*,#58232,.T.);
#86187=ORIENTED_EDGE('',*,*,#58230,.T.);
#86188=ORIENTED_EDGE('',*,*,#58225,.T.);
#86189=ORIENTED_EDGE('',*,*,#58478,.T.);
#86190=ORIENTED_EDGE('',*,*,#58479,.T.);
#86191=ORIENTED_EDGE('',*,*,#58480,.T.);
#86192=ORIENTED_EDGE('',*,*,#58481,.T.);
#86193=ORIENTED_EDGE('',*,*,#58482,.T.);
#86194=ORIENTED_EDGE('',*,*,#58330,.T.);
#86195=ORIENTED_EDGE('',*,*,#58344,.T.);
#86196=ORIENTED_EDGE('',*,*,#58347,.T.);
#86197=ORIENTED_EDGE('',*,*,#58350,.T.);
#86198=ORIENTED_EDGE('',*,*,#58353,.T.);
#86199=ORIENTED_EDGE('',*,*,#58356,.T.);
#86200=ORIENTED_EDGE('',*,*,#58359,.T.);
#86201=ORIENTED_EDGE('',*,*,#58362,.T.);
#86202=ORIENTED_EDGE('',*,*,#58364,.T.);
#86203=ORIENTED_EDGE('',*,*,#58251,.F.);
#86204=ORIENTED_EDGE('',*,*,#58254,.F.);
#86205=ORIENTED_EDGE('',*,*,#58257,.F.);
#86206=ORIENTED_EDGE('',*,*,#58260,.F.);
#86207=ORIENTED_EDGE('',*,*,#58263,.F.);
#86208=ORIENTED_EDGE('',*,*,#58249,.T.);
#86209=ORIENTED_EDGE('',*,*,#58202,.F.);
#86210=ORIENTED_EDGE('',*,*,#58308,.T.);
#86211=ORIENTED_EDGE('',*,*,#58317,.T.);
#86212=ORIENTED_EDGE('',*,*,#58298,.T.);
#86213=ORIENTED_EDGE('',*,*,#58339,.T.);
#86214=ORIENTED_EDGE('',*,*,#58333,.T.);
#86215=ORIENTED_EDGE('',*,*,#58321,.T.);
#86216=ORIENTED_EDGE('',*,*,#58326,.T.);
#86217=ORIENTED_EDGE('',*,*,#58315,.T.);
#86218=ORIENTED_EDGE('',*,*,#58363,.F.);
#86219=ORIENTED_EDGE('',*,*,#58360,.F.);
#86220=ORIENTED_EDGE('',*,*,#58357,.F.);
#86221=ORIENTED_EDGE('',*,*,#58354,.F.);
#86222=ORIENTED_EDGE('',*,*,#58351,.F.);
#86223=ORIENTED_EDGE('',*,*,#58348,.F.);
#86224=ORIENTED_EDGE('',*,*,#58345,.F.);
#86225=ORIENTED_EDGE('',*,*,#58342,.F.);
#86226=ORIENTED_EDGE('',*,*,#58394,.F.);
#86227=ORIENTED_EDGE('',*,*,#58483,.T.);
#86228=ORIENTED_EDGE('',*,*,#58291,.F.);
#86229=ORIENTED_EDGE('',*,*,#58484,.T.);
#86230=ORIENTED_EDGE('',*,*,#58268,.F.);
#86231=ORIENTED_EDGE('',*,*,#58485,.T.);
#86232=ORIENTED_EDGE('',*,*,#58407,.F.);
#86233=ORIENTED_EDGE('',*,*,#58486,.T.);
#86234=ORIENTED_EDGE('',*,*,#58279,.F.);
#86235=ORIENTED_EDGE('',*,*,#58487,.T.);
#86236=ORIENTED_EDGE('',*,*,#58422,.F.);
#86237=ORIENTED_EDGE('',*,*,#58488,.T.);
#86238=ORIENTED_EDGE('',*,*,#58285,.F.);
#86239=ORIENTED_EDGE('',*,*,#58489,.T.);
#86240=ORIENTED_EDGE('',*,*,#58265,.F.);
#86241=ORIENTED_EDGE('',*,*,#58490,.T.);
#86242=ORIENTED_EDGE('',*,*,#58491,.F.);
#86243=ORIENTED_EDGE('',*,*,#58492,.T.);
#86244=ORIENTED_EDGE('',*,*,#58451,.F.);
#86245=ORIENTED_EDGE('',*,*,#58493,.T.);
#86246=ORIENTED_EDGE('',*,*,#58419,.F.);
#86247=ORIENTED_EDGE('',*,*,#58487,.F.);
#86248=ORIENTED_EDGE('',*,*,#58494,.T.);
#86249=ORIENTED_EDGE('',*,*,#58495,.T.);
#86250=ORIENTED_EDGE('',*,*,#58491,.T.);
#86251=ORIENTED_EDGE('',*,*,#58467,.F.);
#86252=ORIENTED_EDGE('',*,*,#58496,.T.);
#86253=ORIENTED_EDGE('',*,*,#58497,.F.);
#86254=ORIENTED_EDGE('',*,*,#58421,.F.);
#86255=ORIENTED_EDGE('',*,*,#58498,.T.);
#86256=ORIENTED_EDGE('',*,*,#58499,.T.);
#86257=ORIENTED_EDGE('',*,*,#58500,.T.);
#86258=ORIENTED_EDGE('',*,*,#58488,.F.);
#86259=ORIENTED_EDGE('',*,*,#58497,.T.);
#86260=ORIENTED_EDGE('',*,*,#58501,.F.);
#86261=ORIENTED_EDGE('',*,*,#58502,.T.);
#86262=ORIENTED_EDGE('',*,*,#58469,.F.);
#86263=ORIENTED_EDGE('',*,*,#58227,.T.);
#86264=ORIENTED_EDGE('',*,*,#58266,.F.);
#86265=ORIENTED_EDGE('',*,*,#58489,.F.);
#86266=ORIENTED_EDGE('',*,*,#58503,.T.);
#86267=ORIENTED_EDGE('',*,*,#58504,.T.);
#86268=ORIENTED_EDGE('',*,*,#58501,.T.);
#86269=ORIENTED_EDGE('',*,*,#58481,.F.);
#86270=ORIENTED_EDGE('',*,*,#58505,.T.);
#86271=ORIENTED_EDGE('',*,*,#58506,.T.);
#86272=ORIENTED_EDGE('',*,*,#58507,.F.);
#86273=ORIENTED_EDGE('',*,*,#58264,.F.);
#86274=ORIENTED_EDGE('',*,*,#58234,.T.);
#86275=ORIENTED_EDGE('',*,*,#58508,.T.);
#86276=ORIENTED_EDGE('',*,*,#58509,.T.);
#86277=ORIENTED_EDGE('',*,*,#58490,.F.);
#86278=ORIENTED_EDGE('',*,*,#58507,.T.);
#86279=ORIENTED_EDGE('',*,*,#58510,.F.);
#86280=ORIENTED_EDGE('',*,*,#58511,.T.);
#86281=ORIENTED_EDGE('',*,*,#58429,.F.);
#86282=ORIENTED_EDGE('',*,*,#58399,.F.);
#86283=ORIENTED_EDGE('',*,*,#58395,.F.);
#86284=ORIENTED_EDGE('',*,*,#58484,.F.);
#86285=ORIENTED_EDGE('',*,*,#58512,.T.);
#86286=ORIENTED_EDGE('',*,*,#58513,.T.);
#86287=ORIENTED_EDGE('',*,*,#58510,.T.);
#86288=ORIENTED_EDGE('',*,*,#58436,.F.);
#86289=ORIENTED_EDGE('',*,*,#58514,.T.);
#86290=ORIENTED_EDGE('',*,*,#58515,.F.);
#86291=ORIENTED_EDGE('',*,*,#58409,.F.);
#86292=ORIENTED_EDGE('',*,*,#58405,.F.);
#86293=ORIENTED_EDGE('',*,*,#58516,.T.);
#86294=ORIENTED_EDGE('',*,*,#58517,.T.);
#86295=ORIENTED_EDGE('',*,*,#58486,.F.);
#86296=ORIENTED_EDGE('',*,*,#58515,.T.);
#86297=ORIENTED_EDGE('',*,*,#58518,.T.);
#86298=ORIENTED_EDGE('',*,*,#58519,.T.);
#86299=ORIENTED_EDGE('',*,*,#58248,.F.);
#86300=ORIENTED_EDGE('',*,*,#58243,.T.);
#86301=ORIENTED_EDGE('',*,*,#58246,.F.);
#86302=ORIENTED_EDGE('',*,*,#58520,.T.);
#86303=ORIENTED_EDGE('',*,*,#58521,.T.);
#86304=ORIENTED_EDGE('',*,*,#58236,.T.);
#86305=ORIENTED_EDGE('',*,*,#58522,.F.);
#86306=ORIENTED_EDGE('',*,*,#58460,.F.);
#86307=ORIENTED_EDGE('',*,*,#58523,.F.);
#86308=ORIENTED_EDGE('',*,*,#58498,.F.);
#86309=ORIENTED_EDGE('',*,*,#58523,.T.);
#86310=ORIENTED_EDGE('',*,*,#58459,.F.);
#86311=ORIENTED_EDGE('',*,*,#58524,.F.);
#86312=ORIENTED_EDGE('',*,*,#58468,.F.);
#86313=ORIENTED_EDGE('',*,*,#58522,.T.);
#86314=ORIENTED_EDGE('',*,*,#58420,.F.);
#86315=ORIENTED_EDGE('',*,*,#58525,.F.);
#86316=ORIENTED_EDGE('',*,*,#58461,.F.);
#86317=ORIENTED_EDGE('',*,*,#58524,.T.);
#86318=ORIENTED_EDGE('',*,*,#58458,.F.);
#86319=ORIENTED_EDGE('',*,*,#58526,.F.);
#86320=ORIENTED_EDGE('',*,*,#58324,.F.);
#86321=ORIENTED_EDGE('',*,*,#58525,.T.);
#86322=ORIENTED_EDGE('',*,*,#58493,.F.);
#86323=ORIENTED_EDGE('',*,*,#58527,.F.);
#86324=ORIENTED_EDGE('',*,*,#58462,.F.);
#86325=ORIENTED_EDGE('',*,*,#58325,.F.);
#86326=ORIENTED_EDGE('',*,*,#58526,.T.);
#86327=ORIENTED_EDGE('',*,*,#58528,.F.);
#86328=ORIENTED_EDGE('',*,*,#58527,.T.);
#86329=ORIENTED_EDGE('',*,*,#58455,.F.);
#86330=ORIENTED_EDGE('',*,*,#58529,.F.);
#86331=ORIENTED_EDGE('',*,*,#58463,.F.);
#86332=ORIENTED_EDGE('',*,*,#58528,.T.);
#86333=ORIENTED_EDGE('',*,*,#58457,.F.);
#86334=ORIENTED_EDGE('',*,*,#58530,.F.);
#86335=ORIENTED_EDGE('',*,*,#58314,.F.);
#86336=ORIENTED_EDGE('',*,*,#58529,.T.);
#86337=ORIENTED_EDGE('',*,*,#58311,.F.);
#86338=ORIENTED_EDGE('',*,*,#58531,.F.);
#86339=ORIENTED_EDGE('',*,*,#58456,.F.);
#86340=ORIENTED_EDGE('',*,*,#58310,.F.);
#86341=ORIENTED_EDGE('',*,*,#58530,.T.);
#86342=ORIENTED_EDGE('',*,*,#58531,.T.);
#86343=ORIENTED_EDGE('',*,*,#58233,.T.);
#86344=ORIENTED_EDGE('',*,*,#58477,.F.);
#86345=ORIENTED_EDGE('',*,*,#58532,.F.);
#86346=ORIENTED_EDGE('',*,*,#58482,.F.);
#86347=ORIENTED_EDGE('',*,*,#58532,.T.);
#86348=ORIENTED_EDGE('',*,*,#58476,.F.);
#86349=ORIENTED_EDGE('',*,*,#58533,.F.);
#86350=ORIENTED_EDGE('',*,*,#58331,.F.);
#86351=ORIENTED_EDGE('',*,*,#58332,.F.);
#86352=ORIENTED_EDGE('',*,*,#58533,.T.);
#86353=ORIENTED_EDGE('',*,*,#58534,.F.);
#86354=ORIENTED_EDGE('',*,*,#58228,.T.);
#86355=ORIENTED_EDGE('',*,*,#58473,.F.);
#86356=ORIENTED_EDGE('',*,*,#58535,.F.);
#86357=ORIENTED_EDGE('',*,*,#58478,.F.);
#86358=ORIENTED_EDGE('',*,*,#58534,.T.);
#86359=ORIENTED_EDGE('',*,*,#58475,.F.);
#86360=ORIENTED_EDGE('',*,*,#58536,.F.);
#86361=ORIENTED_EDGE('',*,*,#58319,.F.);
#86362=ORIENTED_EDGE('',*,*,#58535,.T.);
#86363=ORIENTED_EDGE('',*,*,#58328,.F.);
#86364=ORIENTED_EDGE('',*,*,#58537,.F.);
#86365=ORIENTED_EDGE('',*,*,#58474,.F.);
#86366=ORIENTED_EDGE('',*,*,#58327,.F.);
#86367=ORIENTED_EDGE('',*,*,#58536,.T.);
#86368=ORIENTED_EDGE('',*,*,#58537,.T.);
#86369=ORIENTED_EDGE('',*,*,#58222,.T.);
#86370=ORIENTED_EDGE('',*,*,#58444,.F.);
#86371=ORIENTED_EDGE('',*,*,#58538,.F.);
#86372=ORIENTED_EDGE('',*,*,#58450,.F.);
#86373=ORIENTED_EDGE('',*,*,#58224,.T.);
#86374=ORIENTED_EDGE('',*,*,#58414,.F.);
#86375=ORIENTED_EDGE('',*,*,#58218,.F.);
#86376=ORIENTED_EDGE('',*,*,#58445,.F.);
#86377=ORIENTED_EDGE('',*,*,#58538,.T.);
#86378=ORIENTED_EDGE('',*,*,#58443,.F.);
#86379=ORIENTED_EDGE('',*,*,#58539,.F.);
#86380=ORIENTED_EDGE('',*,*,#58305,.F.);
#86381=ORIENTED_EDGE('',*,*,#58306,.F.);
#86382=ORIENTED_EDGE('',*,*,#58539,.T.);
#86383=ORIENTED_EDGE('',*,*,#58540,.F.);
#86384=ORIENTED_EDGE('',*,*,#58220,.T.);
#86385=ORIENTED_EDGE('',*,*,#58440,.F.);
#86386=ORIENTED_EDGE('',*,*,#58541,.F.);
#86387=ORIENTED_EDGE('',*,*,#58446,.F.);
#86388=ORIENTED_EDGE('',*,*,#58540,.T.);
#86389=ORIENTED_EDGE('',*,*,#58442,.F.);
#86390=ORIENTED_EDGE('',*,*,#58542,.F.);
#86391=ORIENTED_EDGE('',*,*,#58316,.F.);
#86392=ORIENTED_EDGE('',*,*,#58541,.T.);
#86393=ORIENTED_EDGE('',*,*,#58301,.F.);
#86394=ORIENTED_EDGE('',*,*,#58543,.F.);
#86395=ORIENTED_EDGE('',*,*,#58441,.F.);
#86396=ORIENTED_EDGE('',*,*,#58300,.F.);
#86397=ORIENTED_EDGE('',*,*,#58542,.T.);
#86398=ORIENTED_EDGE('',*,*,#58543,.T.);
#86399=ORIENTED_EDGE('',*,*,#58403,.F.);
#86400=ORIENTED_EDGE('',*,*,#58544,.T.);
#86401=ORIENTED_EDGE('',*,*,#58340,.F.);
#86402=ORIENTED_EDGE('',*,*,#58296,.F.);
#86403=ORIENTED_EDGE('',*,*,#58390,.F.);
#86404=ORIENTED_EDGE('',*,*,#58545,.T.);
#86405=ORIENTED_EDGE('',*,*,#58337,.F.);
#86406=ORIENTED_EDGE('',*,*,#58546,.T.);
#86407=ORIENTED_EDGE('',*,*,#58338,.F.);
#86408=ORIENTED_EDGE('',*,*,#58547,.T.);
#86409=ORIENTED_EDGE('',*,*,#58396,.F.);
#86410=ORIENTED_EDGE('',*,*,#58335,.F.);
#86411=ORIENTED_EDGE('',*,*,#58439,.F.);
#86412=ORIENTED_EDGE('',*,*,#58548,.T.);
#86413=ORIENTED_EDGE('',*,*,#58410,.F.);
#86414=ORIENTED_EDGE('',*,*,#58549,.F.);
#86415=ORIENTED_EDGE('',*,*,#58549,.T.);
#86416=ORIENTED_EDGE('',*,*,#58413,.F.);
#86417=ORIENTED_EDGE('',*,*,#58550,.F.);
#86418=ORIENTED_EDGE('',*,*,#58293,.F.);
#86419=ORIENTED_EDGE('',*,*,#58412,.F.);
#86420=ORIENTED_EDGE('',*,*,#58551,.T.);
#86421=ORIENTED_EDGE('',*,*,#58433,.F.);
#86422=ORIENTED_EDGE('',*,*,#58550,.T.);
#86423=ORIENTED_EDGE('',*,*,#58432,.F.);
#86424=ORIENTED_EDGE('',*,*,#58552,.T.);
#86425=ORIENTED_EDGE('',*,*,#58426,.F.);
#86426=ORIENTED_EDGE('',*,*,#58214,.F.);
#86427=ORIENTED_EDGE('',*,*,#58428,.F.);
#86428=ORIENTED_EDGE('',*,*,#58553,.T.);
#86429=ORIENTED_EDGE('',*,*,#58479,.F.);
#86430=ORIENTED_EDGE('',*,*,#58216,.T.);
#86431=ORIENTED_EDGE('',*,*,#58472,.F.);
#86432=ORIENTED_EDGE('',*,*,#58554,.T.);
#86433=ORIENTED_EDGE('',*,*,#58423,.F.);
#86434=ORIENTED_EDGE('',*,*,#58210,.F.);
#86435=ORIENTED_EDGE('',*,*,#58425,.F.);
#86436=ORIENTED_EDGE('',*,*,#58555,.T.);
#86437=ORIENTED_EDGE('',*,*,#58464,.F.);
#86438=ORIENTED_EDGE('',*,*,#58212,.T.);
#86439=ORIENTED_EDGE('',*,*,#58454,.F.);
#86440=ORIENTED_EDGE('',*,*,#58556,.T.);
#86441=ORIENTED_EDGE('',*,*,#58415,.F.);
#86442=ORIENTED_EDGE('',*,*,#58557,.F.);
#86443=ORIENTED_EDGE('',*,*,#58557,.T.);
#86444=ORIENTED_EDGE('',*,*,#58418,.F.);
#86445=ORIENTED_EDGE('',*,*,#58558,.F.);
#86446=ORIENTED_EDGE('',*,*,#58303,.F.);
#86447=ORIENTED_EDGE('',*,*,#58417,.F.);
#86448=ORIENTED_EDGE('',*,*,#58559,.T.);
#86449=ORIENTED_EDGE('',*,*,#58447,.F.);
#86450=ORIENTED_EDGE('',*,*,#58558,.T.);
#86451=ORIENTED_EDGE('',*,*,#58560,.T.);
#86452=ORIENTED_EDGE('',*,*,#58561,.T.);
#86453=ORIENTED_EDGE('',*,*,#58277,.F.);
#86454=ORIENTED_EDGE('',*,*,#58562,.F.);
#86455=ORIENTED_EDGE('',*,*,#58556,.F.);
#86456=ORIENTED_EDGE('',*,*,#58453,.F.);
#86457=ORIENTED_EDGE('',*,*,#58562,.T.);
#86458=ORIENTED_EDGE('',*,*,#58276,.F.);
#86459=ORIENTED_EDGE('',*,*,#58563,.F.);
#86460=ORIENTED_EDGE('',*,*,#58416,.F.);
#86461=ORIENTED_EDGE('',*,*,#58275,.F.);
#86462=ORIENTED_EDGE('',*,*,#58564,.T.);
#86463=ORIENTED_EDGE('',*,*,#58565,.T.);
#86464=ORIENTED_EDGE('',*,*,#58448,.F.);
#86465=ORIENTED_EDGE('',*,*,#58559,.F.);
#86466=ORIENTED_EDGE('',*,*,#58563,.T.);
#86467=ORIENTED_EDGE('',*,*,#58566,.T.);
#86468=ORIENTED_EDGE('',*,*,#58567,.T.);
#86469=ORIENTED_EDGE('',*,*,#58283,.F.);
#86470=ORIENTED_EDGE('',*,*,#58568,.F.);
#86471=ORIENTED_EDGE('',*,*,#58554,.F.);
#86472=ORIENTED_EDGE('',*,*,#58471,.F.);
#86473=ORIENTED_EDGE('',*,*,#58568,.T.);
#86474=ORIENTED_EDGE('',*,*,#58282,.F.);
#86475=ORIENTED_EDGE('',*,*,#58569,.F.);
#86476=ORIENTED_EDGE('',*,*,#58424,.F.);
#86477=ORIENTED_EDGE('',*,*,#58570,.T.);
#86478=ORIENTED_EDGE('',*,*,#58571,.T.);
#86479=ORIENTED_EDGE('',*,*,#58465,.F.);
#86480=ORIENTED_EDGE('',*,*,#58555,.F.);
#86481=ORIENTED_EDGE('',*,*,#58569,.T.);
#86482=ORIENTED_EDGE('',*,*,#58281,.F.);
#86483=ORIENTED_EDGE('',*,*,#58572,.T.);
#86484=ORIENTED_EDGE('',*,*,#58573,.T.);
#86485=ORIENTED_EDGE('',*,*,#58289,.F.);
#86486=ORIENTED_EDGE('',*,*,#58574,.F.);
#86487=ORIENTED_EDGE('',*,*,#58552,.F.);
#86488=ORIENTED_EDGE('',*,*,#58431,.F.);
#86489=ORIENTED_EDGE('',*,*,#58574,.T.);
#86490=ORIENTED_EDGE('',*,*,#58288,.F.);
#86491=ORIENTED_EDGE('',*,*,#58575,.F.);
#86492=ORIENTED_EDGE('',*,*,#58427,.F.);
#86493=ORIENTED_EDGE('',*,*,#58287,.F.);
#86494=ORIENTED_EDGE('',*,*,#58576,.T.);
#86495=ORIENTED_EDGE('',*,*,#58577,.T.);
#86496=ORIENTED_EDGE('',*,*,#58578,.T.);
#86497=ORIENTED_EDGE('',*,*,#58553,.F.);
#86498=ORIENTED_EDGE('',*,*,#58575,.T.);
#86499=ORIENTED_EDGE('',*,*,#58270,.F.);
#86500=ORIENTED_EDGE('',*,*,#58579,.T.);
#86501=ORIENTED_EDGE('',*,*,#58580,.T.);
#86502=ORIENTED_EDGE('',*,*,#58434,.F.);
#86503=ORIENTED_EDGE('',*,*,#58551,.F.);
#86504=ORIENTED_EDGE('',*,*,#58581,.F.);
#86505=ORIENTED_EDGE('',*,*,#58581,.T.);
#86506=ORIENTED_EDGE('',*,*,#58411,.F.);
#86507=ORIENTED_EDGE('',*,*,#58582,.F.);
#86508=ORIENTED_EDGE('',*,*,#58271,.F.);
#86509=ORIENTED_EDGE('',*,*,#58583,.T.);
#86510=ORIENTED_EDGE('',*,*,#58584,.T.);
#86511=ORIENTED_EDGE('',*,*,#58272,.F.);
#86512=ORIENTED_EDGE('',*,*,#58582,.T.);
#86513=ORIENTED_EDGE('',*,*,#58548,.F.);
#86514=ORIENTED_EDGE('',*,*,#58438,.F.);
#86515=ORIENTED_EDGE('',*,*,#58380,.F.);
#86516=ORIENTED_EDGE('',*,*,#58585,.T.);
#86517=ORIENTED_EDGE('',*,*,#58292,.F.);
#86518=ORIENTED_EDGE('',*,*,#58586,.F.);
#86519=ORIENTED_EDGE('',*,*,#58586,.T.);
#86520=ORIENTED_EDGE('',*,*,#58483,.F.);
#86521=ORIENTED_EDGE('',*,*,#58587,.F.);
#86522=ORIENTED_EDGE('',*,*,#58381,.F.);
#86523=ORIENTED_EDGE('',*,*,#58587,.T.);
#86524=ORIENTED_EDGE('',*,*,#58393,.F.);
#86525=ORIENTED_EDGE('',*,*,#58398,.F.);
#86526=ORIENTED_EDGE('',*,*,#58588,.T.);
#86527=ORIENTED_EDGE('',*,*,#58382,.F.);
#86528=ORIENTED_EDGE('',*,*,#58267,.F.);
#86529=ORIENTED_EDGE('',*,*,#58589,.T.);
#86530=ORIENTED_EDGE('',*,*,#58370,.F.);
#86531=ORIENTED_EDGE('',*,*,#58590,.F.);
#86532=ORIENTED_EDGE('',*,*,#58590,.T.);
#86533=ORIENTED_EDGE('',*,*,#58377,.F.);
#86534=ORIENTED_EDGE('',*,*,#58591,.F.);
#86535=ORIENTED_EDGE('',*,*,#58485,.F.);
#86536=ORIENTED_EDGE('',*,*,#58591,.T.);
#86537=ORIENTED_EDGE('',*,*,#58376,.F.);
#86538=ORIENTED_EDGE('',*,*,#58592,.T.);
#86539=ORIENTED_EDGE('',*,*,#58401,.F.);
#86540=ORIENTED_EDGE('',*,*,#58408,.F.);
#86541=ORIENTED_EDGE('',*,*,#58593,.F.);
#86542=ORIENTED_EDGE('',*,*,#58389,.F.);
#86543=ORIENTED_EDGE('',*,*,#58383,.F.);
#86544=ORIENTED_EDGE('',*,*,#58588,.F.);
#86545=ORIENTED_EDGE('',*,*,#58397,.F.);
#86546=ORIENTED_EDGE('',*,*,#58547,.F.);
#86547=ORIENTED_EDGE('',*,*,#58545,.F.);
#86548=ORIENTED_EDGE('',*,*,#58593,.T.);
#86549=ORIENTED_EDGE('',*,*,#58594,.F.);
#86550=ORIENTED_EDGE('',*,*,#58402,.F.);
#86551=ORIENTED_EDGE('',*,*,#58592,.F.);
#86552=ORIENTED_EDGE('',*,*,#58375,.F.);
#86553=ORIENTED_EDGE('',*,*,#58391,.F.);
#86554=ORIENTED_EDGE('',*,*,#58546,.F.);
#86555=ORIENTED_EDGE('',*,*,#58544,.F.);
#86556=ORIENTED_EDGE('',*,*,#58594,.T.);
#86557=ORIENTED_EDGE('',*,*,#58385,.F.);
#86558=ORIENTED_EDGE('',*,*,#58388,.F.);
#86559=ORIENTED_EDGE('',*,*,#58373,.F.);
#86560=ORIENTED_EDGE('',*,*,#58387,.F.);
#86561=ORIENTED_EDGE('',*,*,#58595,.F.);
#86562=ORIENTED_EDGE('',*,*,#58480,.F.);
#86563=ORIENTED_EDGE('',*,*,#58578,.F.);
#86564=ORIENTED_EDGE('',*,*,#58505,.F.);
#86565=ORIENTED_EDGE('',*,*,#58595,.T.);
#86566=ORIENTED_EDGE('',*,*,#58596,.F.);
#86567=ORIENTED_EDGE('',*,*,#58596,.T.);
#86568=ORIENTED_EDGE('',*,*,#58577,.F.);
#86569=ORIENTED_EDGE('',*,*,#58597,.F.);
#86570=ORIENTED_EDGE('',*,*,#58506,.F.);
#86571=ORIENTED_EDGE('',*,*,#58597,.T.);
#86572=ORIENTED_EDGE('',*,*,#58576,.F.);
#86573=ORIENTED_EDGE('',*,*,#58598,.F.);
#86574=ORIENTED_EDGE('',*,*,#58508,.F.);
#86575=ORIENTED_EDGE('',*,*,#58286,.F.);
#86576=ORIENTED_EDGE('',*,*,#58509,.F.);
#86577=ORIENTED_EDGE('',*,*,#58598,.T.);
#86578=ORIENTED_EDGE('',*,*,#58430,.F.);
#86579=ORIENTED_EDGE('',*,*,#58511,.F.);
#86580=ORIENTED_EDGE('',*,*,#58599,.F.);
#86581=ORIENTED_EDGE('',*,*,#58572,.F.);
#86582=ORIENTED_EDGE('',*,*,#58599,.T.);
#86583=ORIENTED_EDGE('',*,*,#58513,.F.);
#86584=ORIENTED_EDGE('',*,*,#58600,.F.);
#86585=ORIENTED_EDGE('',*,*,#58573,.F.);
#86586=ORIENTED_EDGE('',*,*,#58600,.T.);
#86587=ORIENTED_EDGE('',*,*,#58512,.F.);
#86588=ORIENTED_EDGE('',*,*,#58290,.F.);
#86589=ORIENTED_EDGE('',*,*,#58435,.F.);
#86590=ORIENTED_EDGE('',*,*,#58580,.F.);
#86591=ORIENTED_EDGE('',*,*,#58601,.F.);
#86592=ORIENTED_EDGE('',*,*,#58514,.F.);
#86593=ORIENTED_EDGE('',*,*,#58601,.T.);
#86594=ORIENTED_EDGE('',*,*,#58579,.F.);
#86595=ORIENTED_EDGE('',*,*,#58602,.F.);
#86596=ORIENTED_EDGE('',*,*,#58516,.F.);
#86597=ORIENTED_EDGE('',*,*,#58269,.F.);
#86598=ORIENTED_EDGE('',*,*,#58517,.F.);
#86599=ORIENTED_EDGE('',*,*,#58602,.T.);
#86600=ORIENTED_EDGE('',*,*,#58437,.F.);
#86601=ORIENTED_EDGE('',*,*,#58238,.F.);
#86602=ORIENTED_EDGE('',*,*,#58237,.F.);
#86603=ORIENTED_EDGE('',*,*,#58603,.F.);
#86604=ORIENTED_EDGE('',*,*,#58583,.F.);
#86605=ORIENTED_EDGE('',*,*,#58603,.T.);
#86606=ORIENTED_EDGE('',*,*,#58521,.F.);
#86607=ORIENTED_EDGE('',*,*,#58604,.F.);
#86608=ORIENTED_EDGE('',*,*,#58584,.F.);
#86609=ORIENTED_EDGE('',*,*,#58604,.T.);
#86610=ORIENTED_EDGE('',*,*,#58520,.F.);
#86611=ORIENTED_EDGE('',*,*,#58273,.F.);
#86612=ORIENTED_EDGE('',*,*,#58449,.F.);
#86613=ORIENTED_EDGE('',*,*,#58565,.F.);
#86614=ORIENTED_EDGE('',*,*,#58605,.F.);
#86615=ORIENTED_EDGE('',*,*,#58242,.F.);
#86616=ORIENTED_EDGE('',*,*,#58241,.F.);
#86617=ORIENTED_EDGE('',*,*,#58605,.T.);
#86618=ORIENTED_EDGE('',*,*,#58564,.F.);
#86619=ORIENTED_EDGE('',*,*,#58606,.F.);
#86620=ORIENTED_EDGE('',*,*,#58518,.F.);
#86621=ORIENTED_EDGE('',*,*,#58274,.F.);
#86622=ORIENTED_EDGE('',*,*,#58519,.F.);
#86623=ORIENTED_EDGE('',*,*,#58606,.T.);
#86624=ORIENTED_EDGE('',*,*,#58452,.F.);
#86625=ORIENTED_EDGE('',*,*,#58492,.F.);
#86626=ORIENTED_EDGE('',*,*,#58607,.F.);
#86627=ORIENTED_EDGE('',*,*,#58560,.F.);
#86628=ORIENTED_EDGE('',*,*,#58607,.T.);
#86629=ORIENTED_EDGE('',*,*,#58495,.F.);
#86630=ORIENTED_EDGE('',*,*,#58608,.F.);
#86631=ORIENTED_EDGE('',*,*,#58561,.F.);
#86632=ORIENTED_EDGE('',*,*,#58608,.T.);
#86633=ORIENTED_EDGE('',*,*,#58494,.F.);
#86634=ORIENTED_EDGE('',*,*,#58278,.F.);
#86635=ORIENTED_EDGE('',*,*,#58280,.F.);
#86636=ORIENTED_EDGE('',*,*,#58500,.F.);
#86637=ORIENTED_EDGE('',*,*,#58609,.F.);
#86638=ORIENTED_EDGE('',*,*,#58609,.T.);
#86639=ORIENTED_EDGE('',*,*,#58499,.F.);
#86640=ORIENTED_EDGE('',*,*,#58610,.F.);
#86641=ORIENTED_EDGE('',*,*,#58570,.F.);
#86642=ORIENTED_EDGE('',*,*,#58466,.F.);
#86643=ORIENTED_EDGE('',*,*,#58571,.F.);
#86644=ORIENTED_EDGE('',*,*,#58610,.T.);
#86645=ORIENTED_EDGE('',*,*,#58496,.F.);
#86646=ORIENTED_EDGE('',*,*,#58470,.F.);
#86647=ORIENTED_EDGE('',*,*,#58502,.F.);
#86648=ORIENTED_EDGE('',*,*,#58611,.F.);
#86649=ORIENTED_EDGE('',*,*,#58566,.F.);
#86650=ORIENTED_EDGE('',*,*,#58611,.T.);
#86651=ORIENTED_EDGE('',*,*,#58504,.F.);
#86652=ORIENTED_EDGE('',*,*,#58612,.F.);
#86653=ORIENTED_EDGE('',*,*,#58567,.F.);
#86654=ORIENTED_EDGE('',*,*,#58612,.T.);
#86655=ORIENTED_EDGE('',*,*,#58503,.F.);
#86656=ORIENTED_EDGE('',*,*,#58284,.F.);
#86657=ORIENTED_EDGE('',*,*,#58613,.F.);
#86658=ORIENTED_EDGE('',*,*,#58589,.F.);
#86659=ORIENTED_EDGE('',*,*,#58208,.F.);
#86660=ORIENTED_EDGE('',*,*,#58369,.F.);
#86661=ORIENTED_EDGE('',*,*,#58613,.T.);
#86662=ORIENTED_EDGE('',*,*,#58368,.F.);
#86663=ORIENTED_EDGE('',*,*,#58614,.F.);
#86664=ORIENTED_EDGE('',*,*,#58371,.F.);
#86665=ORIENTED_EDGE('',*,*,#58206,.T.);
#86666=ORIENTED_EDGE('',*,*,#58585,.F.);
#86667=ORIENTED_EDGE('',*,*,#58615,.F.);
#86668=ORIENTED_EDGE('',*,*,#58365,.F.);
#86669=ORIENTED_EDGE('',*,*,#58614,.T.);
#86670=ORIENTED_EDGE('',*,*,#58367,.F.);
#86671=ORIENTED_EDGE('',*,*,#58616,.F.);
#86672=ORIENTED_EDGE('',*,*,#58386,.F.);
#86673=ORIENTED_EDGE('',*,*,#58615,.T.);
#86674=ORIENTED_EDGE('',*,*,#58379,.F.);
#86675=ORIENTED_EDGE('',*,*,#58616,.T.);
#86676=ORIENTED_EDGE('',*,*,#58366,.F.);
#86677=ORIENTED_EDGE('',*,*,#58617,.T.);
#86678=ORIENTED_EDGE('',*,*,#58617,.F.);
#86679=ORIENTED_EDGE('',*,*,#58618,.F.);
#86680=ORIENTED_EDGE('',*,*,#58619,.T.);
#86681=ORIENTED_EDGE('',*,*,#58620,.F.);
#86682=ORIENTED_EDGE('',*,*,#58619,.F.);
#86683=ORIENTED_EDGE('',*,*,#58621,.F.);
#86684=ORIENTED_EDGE('',*,*,#58622,.F.);
#86685=ORIENTED_EDGE('',*,*,#58623,.T.);
#86686=ORIENTED_EDGE('',*,*,#58624,.F.);
#86687=ORIENTED_EDGE('',*,*,#58623,.F.);
#86688=ORIENTED_EDGE('',*,*,#58625,.F.);
#86689=ORIENTED_EDGE('',*,*,#58626,.F.);
#86690=ORIENTED_EDGE('',*,*,#58627,.T.);
#86691=ORIENTED_EDGE('',*,*,#58628,.F.);
#86692=ORIENTED_EDGE('',*,*,#58629,.F.);
#86693=ORIENTED_EDGE('',*,*,#58630,.F.);
#86694=ORIENTED_EDGE('',*,*,#58631,.F.);
#86695=ORIENTED_EDGE('',*,*,#58632,.T.);
#86696=ORIENTED_EDGE('',*,*,#58629,.T.);
#86697=ORIENTED_EDGE('',*,*,#58628,.T.);
#86698=ORIENTED_EDGE('',*,*,#58633,.T.);
#86699=ORIENTED_EDGE('',*,*,#58634,.T.);
#86700=ORIENTED_EDGE('',*,*,#58635,.T.);
#86701=ORIENTED_EDGE('',*,*,#58636,.T.);
#86702=ORIENTED_EDGE('',*,*,#58626,.T.);
#86703=ORIENTED_EDGE('',*,*,#58631,.T.);
#86704=ORIENTED_EDGE('',*,*,#58637,.T.);
#86705=ORIENTED_EDGE('',*,*,#58635,.F.);
#86706=ORIENTED_EDGE('',*,*,#58622,.T.);
#86707=ORIENTED_EDGE('',*,*,#58638,.T.);
#86708=ORIENTED_EDGE('',*,*,#58621,.T.);
#86709=ORIENTED_EDGE('',*,*,#58618,.T.);
#86710=ORIENTED_EDGE('',*,*,#58638,.F.);
#86711=ORIENTED_EDGE('',*,*,#58625,.T.);
#86712=ORIENTED_EDGE('',*,*,#58620,.T.);
#86713=ORIENTED_EDGE('',*,*,#58639,.F.);
#86714=ORIENTED_EDGE('',*,*,#58639,.T.);
#86715=ORIENTED_EDGE('',*,*,#58624,.T.);
#86716=ORIENTED_EDGE('',*,*,#58634,.F.);
#86717=ORIENTED_EDGE('',*,*,#58627,.F.);
#86718=ORIENTED_EDGE('',*,*,#58636,.F.);
#86719=ORIENTED_EDGE('',*,*,#58637,.F.);
#86720=ORIENTED_EDGE('',*,*,#58630,.T.);
#86721=ORIENTED_EDGE('',*,*,#58632,.F.);
#86722=ORIENTED_EDGE('',*,*,#58633,.F.);
#86723=ORIENTED_EDGE('',*,*,#58640,.F.);
#86724=ORIENTED_EDGE('',*,*,#58641,.T.);
#86725=ORIENTED_EDGE('',*,*,#58642,.F.);
#86726=ORIENTED_EDGE('',*,*,#58641,.F.);
#86727=ORIENTED_EDGE('',*,*,#58643,.F.);
#86728=ORIENTED_EDGE('',*,*,#58644,.F.);
#86729=ORIENTED_EDGE('',*,*,#58645,.T.);
#86730=ORIENTED_EDGE('',*,*,#58646,.F.);
#86731=ORIENTED_EDGE('',*,*,#58647,.F.);
#86732=ORIENTED_EDGE('',*,*,#58645,.F.);
#86733=ORIENTED_EDGE('',*,*,#58648,.F.);
#86734=ORIENTED_EDGE('',*,*,#58649,.T.);
#86735=ORIENTED_EDGE('',*,*,#58650,.T.);
#86736=ORIENTED_EDGE('',*,*,#58651,.T.);
#86737=ORIENTED_EDGE('',*,*,#58649,.F.);
#86738=ORIENTED_EDGE('',*,*,#58652,.F.);
#86739=ORIENTED_EDGE('',*,*,#58653,.T.);
#86740=ORIENTED_EDGE('',*,*,#58643,.T.);
#86741=ORIENTED_EDGE('',*,*,#58640,.T.);
#86742=ORIENTED_EDGE('',*,*,#58653,.F.);
#86743=ORIENTED_EDGE('',*,*,#58648,.T.);
#86744=ORIENTED_EDGE('',*,*,#58646,.T.);
#86745=ORIENTED_EDGE('',*,*,#58647,.T.);
#86746=ORIENTED_EDGE('',*,*,#58654,.T.);
#86747=ORIENTED_EDGE('',*,*,#58655,.T.);
#86748=ORIENTED_EDGE('',*,*,#58654,.F.);
#86749=ORIENTED_EDGE('',*,*,#58651,.F.);
#86750=ORIENTED_EDGE('',*,*,#58650,.F.);
#86751=ORIENTED_EDGE('',*,*,#58655,.F.);
#86752=ORIENTED_EDGE('',*,*,#58652,.T.);
#86753=ORIENTED_EDGE('',*,*,#58644,.T.);
#86754=ORIENTED_EDGE('',*,*,#58642,.T.);
#86755=ORIENTED_EDGE('',*,*,#58656,.F.);
#86756=ORIENTED_EDGE('',*,*,#58657,.T.);
#86757=ORIENTED_EDGE('',*,*,#58658,.F.);
#86758=ORIENTED_EDGE('',*,*,#58657,.F.);
#86759=ORIENTED_EDGE('',*,*,#58659,.F.);
#86760=ORIENTED_EDGE('',*,*,#58660,.T.);
#86761=ORIENTED_EDGE('',*,*,#58661,.F.);
#86762=ORIENTED_EDGE('',*,*,#58662,.F.);
#86763=ORIENTED_EDGE('',*,*,#58660,.F.);
#86764=ORIENTED_EDGE('',*,*,#58663,.F.);
#86765=ORIENTED_EDGE('',*,*,#58664,.F.);
#86766=ORIENTED_EDGE('',*,*,#58665,.T.);
#86767=ORIENTED_EDGE('',*,*,#58666,.F.);
#86768=ORIENTED_EDGE('',*,*,#58665,.F.);
#86769=ORIENTED_EDGE('',*,*,#58667,.F.);
#86770=ORIENTED_EDGE('',*,*,#58668,.T.);
#86771=ORIENTED_EDGE('',*,*,#58669,.F.);
#86772=ORIENTED_EDGE('',*,*,#58668,.F.);
#86773=ORIENTED_EDGE('',*,*,#58670,.F.);
#86774=ORIENTED_EDGE('',*,*,#58671,.T.);
#86775=ORIENTED_EDGE('',*,*,#58672,.F.);
#86776=ORIENTED_EDGE('',*,*,#58671,.F.);
#86777=ORIENTED_EDGE('',*,*,#58673,.F.);
#86778=ORIENTED_EDGE('',*,*,#58674,.T.);
#86779=ORIENTED_EDGE('',*,*,#58675,.T.);
#86780=ORIENTED_EDGE('',*,*,#58674,.F.);
#86781=ORIENTED_EDGE('',*,*,#58658,.T.);
#86782=ORIENTED_EDGE('',*,*,#58676,.T.);
#86783=ORIENTED_EDGE('',*,*,#58667,.T.);
#86784=ORIENTED_EDGE('',*,*,#58676,.F.);
#86785=ORIENTED_EDGE('',*,*,#58672,.T.);
#86786=ORIENTED_EDGE('',*,*,#58677,.T.);
#86787=ORIENTED_EDGE('',*,*,#58673,.T.);
#86788=ORIENTED_EDGE('',*,*,#58677,.F.);
#86789=ORIENTED_EDGE('',*,*,#58678,.T.);
#86790=ORIENTED_EDGE('',*,*,#58679,.T.);
#86791=ORIENTED_EDGE('',*,*,#58661,.T.);
#86792=ORIENTED_EDGE('',*,*,#58662,.T.);
#86793=ORIENTED_EDGE('',*,*,#58679,.F.);
#86794=ORIENTED_EDGE('',*,*,#58663,.T.);
#86795=ORIENTED_EDGE('',*,*,#58664,.T.);
#86796=ORIENTED_EDGE('',*,*,#58680,.T.);
#86797=ORIENTED_EDGE('',*,*,#58681,.T.);
#86798=ORIENTED_EDGE('',*,*,#58680,.F.);
#86799=ORIENTED_EDGE('',*,*,#58682,.F.);
#86800=ORIENTED_EDGE('',*,*,#58683,.T.);
#86801=ORIENTED_EDGE('',*,*,#58684,.T.);
#86802=ORIENTED_EDGE('',*,*,#58683,.F.);
#86803=ORIENTED_EDGE('',*,*,#58684,.F.);
#86804=ORIENTED_EDGE('',*,*,#58675,.F.);
#86805=ORIENTED_EDGE('',*,*,#58682,.T.);
#86806=ORIENTED_EDGE('',*,*,#58681,.F.);
#86807=ORIENTED_EDGE('',*,*,#58659,.T.);
#86808=ORIENTED_EDGE('',*,*,#58666,.T.);
#86809=ORIENTED_EDGE('',*,*,#58670,.T.);
#86810=ORIENTED_EDGE('',*,*,#58669,.T.);
#86811=ORIENTED_EDGE('',*,*,#58656,.T.);
#86812=ORIENTED_EDGE('',*,*,#58678,.F.);
#86813=ORIENTED_EDGE('',*,*,#58685,.F.);
#86814=ORIENTED_EDGE('',*,*,#58686,.T.);
#86815=ORIENTED_EDGE('',*,*,#58687,.T.);
#86816=ORIENTED_EDGE('',*,*,#58688,.F.);
#86817=ORIENTED_EDGE('',*,*,#58689,.F.);
#86818=ORIENTED_EDGE('',*,*,#58690,.T.);
#86819=ORIENTED_EDGE('',*,*,#58685,.T.);
#86820=ORIENTED_EDGE('',*,*,#58691,.F.);
#86821=ORIENTED_EDGE('',*,*,#58692,.F.);
#86822=ORIENTED_EDGE('',*,*,#58693,.T.);
#86823=ORIENTED_EDGE('',*,*,#58689,.T.);
#86824=ORIENTED_EDGE('',*,*,#58694,.F.);
#86825=ORIENTED_EDGE('',*,*,#58695,.F.);
#86826=ORIENTED_EDGE('',*,*,#58696,.T.);
#86827=ORIENTED_EDGE('',*,*,#58692,.T.);
#86828=ORIENTED_EDGE('',*,*,#58697,.F.);
#86829=ORIENTED_EDGE('',*,*,#58698,.F.);
#86830=ORIENTED_EDGE('',*,*,#58699,.T.);
#86831=ORIENTED_EDGE('',*,*,#58695,.T.);
#86832=ORIENTED_EDGE('',*,*,#58700,.F.);
#86833=ORIENTED_EDGE('',*,*,#58701,.F.);
#86834=ORIENTED_EDGE('',*,*,#58702,.T.);
#86835=ORIENTED_EDGE('',*,*,#58698,.T.);
#86836=ORIENTED_EDGE('',*,*,#58703,.F.);
#86837=ORIENTED_EDGE('',*,*,#58704,.F.);
#86838=ORIENTED_EDGE('',*,*,#58705,.F.);
#86839=ORIENTED_EDGE('',*,*,#58706,.T.);
#86840=ORIENTED_EDGE('',*,*,#58707,.F.);
#86841=ORIENTED_EDGE('',*,*,#58708,.F.);
#86842=ORIENTED_EDGE('',*,*,#58704,.T.);
#86843=ORIENTED_EDGE('',*,*,#58709,.T.);
#86844=ORIENTED_EDGE('',*,*,#58710,.F.);
#86845=ORIENTED_EDGE('',*,*,#58711,.F.);
#86846=ORIENTED_EDGE('',*,*,#58712,.F.);
#86847=ORIENTED_EDGE('',*,*,#58707,.T.);
#86848=ORIENTED_EDGE('',*,*,#58713,.F.);
#86849=ORIENTED_EDGE('',*,*,#58714,.F.);
#86850=ORIENTED_EDGE('',*,*,#58715,.F.);
#86851=ORIENTED_EDGE('',*,*,#58711,.T.);
#86852=ORIENTED_EDGE('',*,*,#58716,.F.);
#86853=ORIENTED_EDGE('',*,*,#58717,.F.);
#86854=ORIENTED_EDGE('',*,*,#58718,.F.);
#86855=ORIENTED_EDGE('',*,*,#58714,.T.);
#86856=ORIENTED_EDGE('',*,*,#58719,.F.);
#86857=ORIENTED_EDGE('',*,*,#58720,.F.);
#86858=ORIENTED_EDGE('',*,*,#58721,.F.);
#86859=ORIENTED_EDGE('',*,*,#58717,.T.);
#86860=ORIENTED_EDGE('',*,*,#58722,.F.);
#86861=ORIENTED_EDGE('',*,*,#58723,.F.);
#86862=ORIENTED_EDGE('',*,*,#58724,.F.);
#86863=ORIENTED_EDGE('',*,*,#58720,.T.);
#86864=ORIENTED_EDGE('',*,*,#58725,.F.);
#86865=ORIENTED_EDGE('',*,*,#58726,.F.);
#86866=ORIENTED_EDGE('',*,*,#58727,.T.);
#86867=ORIENTED_EDGE('',*,*,#58728,.F.);
#86868=ORIENTED_EDGE('',*,*,#58723,.T.);
#86869=ORIENTED_EDGE('',*,*,#58729,.F.);
#86870=ORIENTED_EDGE('',*,*,#58706,.F.);
#86871=ORIENTED_EDGE('',*,*,#58730,.F.);
#86872=ORIENTED_EDGE('',*,*,#58731,.F.);
#86873=ORIENTED_EDGE('',*,*,#58732,.F.);
#86874=ORIENTED_EDGE('',*,*,#58709,.F.);
#86875=ORIENTED_EDGE('',*,*,#58733,.T.);
#86876=ORIENTED_EDGE('',*,*,#58734,.F.);
#86877=ORIENTED_EDGE('',*,*,#58733,.F.);
#86878=ORIENTED_EDGE('',*,*,#58735,.F.);
#86879=ORIENTED_EDGE('',*,*,#58736,.F.);
#86880=ORIENTED_EDGE('',*,*,#58687,.F.);
#86881=ORIENTED_EDGE('',*,*,#58737,.F.);
#86882=ORIENTED_EDGE('',*,*,#58727,.F.);
#86883=ORIENTED_EDGE('',*,*,#58738,.F.);
#86884=ORIENTED_EDGE('',*,*,#58739,.T.);
#86885=ORIENTED_EDGE('',*,*,#58740,.F.);
#86886=ORIENTED_EDGE('',*,*,#58739,.F.);
#86887=ORIENTED_EDGE('',*,*,#58726,.T.);
#86888=ORIENTED_EDGE('',*,*,#58741,.F.);
#86889=ORIENTED_EDGE('',*,*,#58735,.T.);
#86890=ORIENTED_EDGE('',*,*,#58738,.T.);
#86891=ORIENTED_EDGE('',*,*,#58734,.T.);
#86892=ORIENTED_EDGE('',*,*,#58740,.T.);
#86893=ORIENTED_EDGE('',*,*,#58742,.F.);
#86894=ORIENTED_EDGE('',*,*,#58743,.F.);
#86895=ORIENTED_EDGE('',*,*,#58744,.F.);
#86896=ORIENTED_EDGE('',*,*,#58745,.F.);
#86897=ORIENTED_EDGE('',*,*,#58746,.F.);
#86898=ORIENTED_EDGE('',*,*,#58747,.F.);
#86899=ORIENTED_EDGE('',*,*,#58742,.T.);
#86900=ORIENTED_EDGE('',*,*,#58748,.F.);
#86901=ORIENTED_EDGE('',*,*,#58747,.T.);
#86902=ORIENTED_EDGE('',*,*,#58749,.F.);
#86903=ORIENTED_EDGE('',*,*,#58746,.T.);
#86904=ORIENTED_EDGE('',*,*,#58750,.F.);
#86905=ORIENTED_EDGE('',*,*,#58745,.T.);
#86906=ORIENTED_EDGE('',*,*,#58751,.F.);
#86907=ORIENTED_EDGE('',*,*,#58744,.T.);
#86908=ORIENTED_EDGE('',*,*,#58752,.F.);
#86909=ORIENTED_EDGE('',*,*,#58743,.T.);
#86910=ORIENTED_EDGE('',*,*,#58753,.F.);
#86911=ORIENTED_EDGE('',*,*,#58754,.T.);
#86912=ORIENTED_EDGE('',*,*,#58755,.T.);
#86913=ORIENTED_EDGE('',*,*,#58756,.T.);
#86914=ORIENTED_EDGE('',*,*,#58757,.T.);
#86915=ORIENTED_EDGE('',*,*,#58758,.T.);
#86916=ORIENTED_EDGE('',*,*,#58759,.T.);
#86917=ORIENTED_EDGE('',*,*,#58760,.T.);
#86918=ORIENTED_EDGE('',*,*,#58748,.T.);
#86919=ORIENTED_EDGE('',*,*,#58761,.F.);
#86920=ORIENTED_EDGE('',*,*,#58755,.F.);
#86921=ORIENTED_EDGE('',*,*,#58761,.T.);
#86922=ORIENTED_EDGE('',*,*,#58749,.T.);
#86923=ORIENTED_EDGE('',*,*,#58762,.F.);
#86924=ORIENTED_EDGE('',*,*,#58756,.F.);
#86925=ORIENTED_EDGE('',*,*,#58762,.T.);
#86926=ORIENTED_EDGE('',*,*,#58750,.T.);
#86927=ORIENTED_EDGE('',*,*,#58763,.F.);
#86928=ORIENTED_EDGE('',*,*,#58757,.F.);
#86929=ORIENTED_EDGE('',*,*,#58763,.T.);
#86930=ORIENTED_EDGE('',*,*,#58751,.T.);
#86931=ORIENTED_EDGE('',*,*,#58764,.F.);
#86932=ORIENTED_EDGE('',*,*,#58758,.F.);
#86933=ORIENTED_EDGE('',*,*,#58764,.T.);
#86934=ORIENTED_EDGE('',*,*,#58752,.T.);
#86935=ORIENTED_EDGE('',*,*,#58765,.F.);
#86936=ORIENTED_EDGE('',*,*,#58759,.F.);
#86937=ORIENTED_EDGE('',*,*,#58765,.T.);
#86938=ORIENTED_EDGE('',*,*,#58753,.T.);
#86939=ORIENTED_EDGE('',*,*,#58760,.F.);
#86940=ORIENTED_EDGE('',*,*,#58754,.F.);
#86941=ORIENTED_EDGE('',*,*,#58736,.T.);
#86942=ORIENTED_EDGE('',*,*,#58741,.T.);
#86943=ORIENTED_EDGE('',*,*,#58729,.T.);
#86944=ORIENTED_EDGE('',*,*,#58725,.T.);
#86945=ORIENTED_EDGE('',*,*,#58722,.T.);
#86946=ORIENTED_EDGE('',*,*,#58719,.T.);
#86947=ORIENTED_EDGE('',*,*,#58716,.T.);
#86948=ORIENTED_EDGE('',*,*,#58713,.T.);
#86949=ORIENTED_EDGE('',*,*,#58710,.T.);
#86950=ORIENTED_EDGE('',*,*,#58732,.T.);
#86951=ORIENTED_EDGE('',*,*,#58766,.T.);
#86952=ORIENTED_EDGE('',*,*,#58703,.T.);
#86953=ORIENTED_EDGE('',*,*,#58700,.T.);
#86954=ORIENTED_EDGE('',*,*,#58697,.T.);
#86955=ORIENTED_EDGE('',*,*,#58694,.T.);
#86956=ORIENTED_EDGE('',*,*,#58691,.T.);
#86957=ORIENTED_EDGE('',*,*,#58688,.T.);
#86958=ORIENTED_EDGE('',*,*,#58701,.T.);
#86959=ORIENTED_EDGE('',*,*,#58766,.F.);
#86960=ORIENTED_EDGE('',*,*,#58731,.T.);
#86961=ORIENTED_EDGE('',*,*,#58767,.T.);
#86962=ORIENTED_EDGE('',*,*,#58737,.T.);
#86963=ORIENTED_EDGE('',*,*,#58686,.F.);
#86964=ORIENTED_EDGE('',*,*,#58690,.F.);
#86965=ORIENTED_EDGE('',*,*,#58693,.F.);
#86966=ORIENTED_EDGE('',*,*,#58696,.F.);
#86967=ORIENTED_EDGE('',*,*,#58699,.F.);
#86968=ORIENTED_EDGE('',*,*,#58702,.F.);
#86969=ORIENTED_EDGE('',*,*,#58767,.F.);
#86970=ORIENTED_EDGE('',*,*,#58730,.T.);
#86971=ORIENTED_EDGE('',*,*,#58705,.T.);
#86972=ORIENTED_EDGE('',*,*,#58708,.T.);
#86973=ORIENTED_EDGE('',*,*,#58712,.T.);
#86974=ORIENTED_EDGE('',*,*,#58715,.T.);
#86975=ORIENTED_EDGE('',*,*,#58718,.T.);
#86976=ORIENTED_EDGE('',*,*,#58721,.T.);
#86977=ORIENTED_EDGE('',*,*,#58724,.T.);
#86978=ORIENTED_EDGE('',*,*,#58728,.T.);
#86979=ORIENTED_EDGE('',*,*,#58768,.F.);
#86980=ORIENTED_EDGE('',*,*,#58769,.T.);
#86981=ORIENTED_EDGE('',*,*,#58770,.T.);
#86982=ORIENTED_EDGE('',*,*,#58771,.F.);
#86983=ORIENTED_EDGE('',*,*,#58772,.F.);
#86984=ORIENTED_EDGE('',*,*,#58773,.T.);
#86985=ORIENTED_EDGE('',*,*,#58768,.T.);
#86986=ORIENTED_EDGE('',*,*,#58774,.F.);
#86987=ORIENTED_EDGE('',*,*,#58775,.F.);
#86988=ORIENTED_EDGE('',*,*,#58776,.T.);
#86989=ORIENTED_EDGE('',*,*,#58772,.T.);
#86990=ORIENTED_EDGE('',*,*,#58777,.F.);
#86991=ORIENTED_EDGE('',*,*,#58778,.F.);
#86992=ORIENTED_EDGE('',*,*,#58779,.T.);
#86993=ORIENTED_EDGE('',*,*,#58775,.T.);
#86994=ORIENTED_EDGE('',*,*,#58780,.F.);
#86995=ORIENTED_EDGE('',*,*,#58781,.F.);
#86996=ORIENTED_EDGE('',*,*,#58782,.T.);
#86997=ORIENTED_EDGE('',*,*,#58778,.T.);
#86998=ORIENTED_EDGE('',*,*,#58783,.F.);
#86999=ORIENTED_EDGE('',*,*,#58784,.F.);
#87000=ORIENTED_EDGE('',*,*,#58785,.T.);
#87001=ORIENTED_EDGE('',*,*,#58781,.T.);
#87002=ORIENTED_EDGE('',*,*,#58786,.F.);
#87003=ORIENTED_EDGE('',*,*,#58787,.F.);
#87004=ORIENTED_EDGE('',*,*,#58788,.F.);
#87005=ORIENTED_EDGE('',*,*,#58789,.T.);
#87006=ORIENTED_EDGE('',*,*,#58790,.F.);
#87007=ORIENTED_EDGE('',*,*,#58791,.F.);
#87008=ORIENTED_EDGE('',*,*,#58787,.T.);
#87009=ORIENTED_EDGE('',*,*,#58792,.T.);
#87010=ORIENTED_EDGE('',*,*,#58793,.F.);
#87011=ORIENTED_EDGE('',*,*,#58794,.F.);
#87012=ORIENTED_EDGE('',*,*,#58795,.F.);
#87013=ORIENTED_EDGE('',*,*,#58790,.T.);
#87014=ORIENTED_EDGE('',*,*,#58796,.F.);
#87015=ORIENTED_EDGE('',*,*,#58797,.F.);
#87016=ORIENTED_EDGE('',*,*,#58798,.F.);
#87017=ORIENTED_EDGE('',*,*,#58794,.T.);
#87018=ORIENTED_EDGE('',*,*,#58799,.F.);
#87019=ORIENTED_EDGE('',*,*,#58800,.F.);
#87020=ORIENTED_EDGE('',*,*,#58801,.F.);
#87021=ORIENTED_EDGE('',*,*,#58797,.T.);
#87022=ORIENTED_EDGE('',*,*,#58802,.F.);
#87023=ORIENTED_EDGE('',*,*,#58803,.F.);
#87024=ORIENTED_EDGE('',*,*,#58804,.F.);
#87025=ORIENTED_EDGE('',*,*,#58800,.T.);
#87026=ORIENTED_EDGE('',*,*,#58805,.F.);
#87027=ORIENTED_EDGE('',*,*,#58806,.F.);
#87028=ORIENTED_EDGE('',*,*,#58807,.F.);
#87029=ORIENTED_EDGE('',*,*,#58803,.T.);
#87030=ORIENTED_EDGE('',*,*,#58808,.F.);
#87031=ORIENTED_EDGE('',*,*,#58809,.F.);
#87032=ORIENTED_EDGE('',*,*,#58810,.T.);
#87033=ORIENTED_EDGE('',*,*,#58811,.F.);
#87034=ORIENTED_EDGE('',*,*,#58806,.T.);
#87035=ORIENTED_EDGE('',*,*,#58812,.F.);
#87036=ORIENTED_EDGE('',*,*,#58789,.F.);
#87037=ORIENTED_EDGE('',*,*,#58813,.F.);
#87038=ORIENTED_EDGE('',*,*,#58814,.F.);
#87039=ORIENTED_EDGE('',*,*,#58815,.F.);
#87040=ORIENTED_EDGE('',*,*,#58792,.F.);
#87041=ORIENTED_EDGE('',*,*,#58816,.T.);
#87042=ORIENTED_EDGE('',*,*,#58817,.F.);
#87043=ORIENTED_EDGE('',*,*,#58816,.F.);
#87044=ORIENTED_EDGE('',*,*,#58818,.F.);
#87045=ORIENTED_EDGE('',*,*,#58819,.F.);
#87046=ORIENTED_EDGE('',*,*,#58770,.F.);
#87047=ORIENTED_EDGE('',*,*,#58820,.F.);
#87048=ORIENTED_EDGE('',*,*,#58810,.F.);
#87049=ORIENTED_EDGE('',*,*,#58821,.F.);
#87050=ORIENTED_EDGE('',*,*,#58822,.T.);
#87051=ORIENTED_EDGE('',*,*,#58823,.F.);
#87052=ORIENTED_EDGE('',*,*,#58822,.F.);
#87053=ORIENTED_EDGE('',*,*,#58809,.T.);
#87054=ORIENTED_EDGE('',*,*,#58824,.F.);
#87055=ORIENTED_EDGE('',*,*,#58818,.T.);
#87056=ORIENTED_EDGE('',*,*,#58821,.T.);
#87057=ORIENTED_EDGE('',*,*,#58817,.T.);
#87058=ORIENTED_EDGE('',*,*,#58823,.T.);
#87059=ORIENTED_EDGE('',*,*,#58825,.F.);
#87060=ORIENTED_EDGE('',*,*,#58826,.F.);
#87061=ORIENTED_EDGE('',*,*,#58827,.F.);
#87062=ORIENTED_EDGE('',*,*,#58828,.F.);
#87063=ORIENTED_EDGE('',*,*,#58829,.F.);
#87064=ORIENTED_EDGE('',*,*,#58830,.F.);
#87065=ORIENTED_EDGE('',*,*,#58825,.T.);
#87066=ORIENTED_EDGE('',*,*,#58831,.F.);
#87067=ORIENTED_EDGE('',*,*,#58830,.T.);
#87068=ORIENTED_EDGE('',*,*,#58832,.F.);
#87069=ORIENTED_EDGE('',*,*,#58829,.T.);
#87070=ORIENTED_EDGE('',*,*,#58833,.F.);
#87071=ORIENTED_EDGE('',*,*,#58828,.T.);
#87072=ORIENTED_EDGE('',*,*,#58834,.F.);
#87073=ORIENTED_EDGE('',*,*,#58827,.T.);
#87074=ORIENTED_EDGE('',*,*,#58835,.F.);
#87075=ORIENTED_EDGE('',*,*,#58826,.T.);
#87076=ORIENTED_EDGE('',*,*,#58836,.F.);
#87077=ORIENTED_EDGE('',*,*,#58837,.T.);
#87078=ORIENTED_EDGE('',*,*,#58838,.T.);
#87079=ORIENTED_EDGE('',*,*,#58839,.T.);
#87080=ORIENTED_EDGE('',*,*,#58840,.T.);
#87081=ORIENTED_EDGE('',*,*,#58841,.T.);
#87082=ORIENTED_EDGE('',*,*,#58842,.T.);
#87083=ORIENTED_EDGE('',*,*,#58843,.T.);
#87084=ORIENTED_EDGE('',*,*,#58831,.T.);
#87085=ORIENTED_EDGE('',*,*,#58844,.F.);
#87086=ORIENTED_EDGE('',*,*,#58838,.F.);
#87087=ORIENTED_EDGE('',*,*,#58844,.T.);
#87088=ORIENTED_EDGE('',*,*,#58832,.T.);
#87089=ORIENTED_EDGE('',*,*,#58845,.F.);
#87090=ORIENTED_EDGE('',*,*,#58839,.F.);
#87091=ORIENTED_EDGE('',*,*,#58845,.T.);
#87092=ORIENTED_EDGE('',*,*,#58833,.T.);
#87093=ORIENTED_EDGE('',*,*,#58846,.F.);
#87094=ORIENTED_EDGE('',*,*,#58840,.F.);
#87095=ORIENTED_EDGE('',*,*,#58846,.T.);
#87096=ORIENTED_EDGE('',*,*,#58834,.T.);
#87097=ORIENTED_EDGE('',*,*,#58847,.F.);
#87098=ORIENTED_EDGE('',*,*,#58841,.F.);
#87099=ORIENTED_EDGE('',*,*,#58847,.T.);
#87100=ORIENTED_EDGE('',*,*,#58835,.T.);
#87101=ORIENTED_EDGE('',*,*,#58848,.F.);
#87102=ORIENTED_EDGE('',*,*,#58842,.F.);
#87103=ORIENTED_EDGE('',*,*,#58848,.T.);
#87104=ORIENTED_EDGE('',*,*,#58836,.T.);
#87105=ORIENTED_EDGE('',*,*,#58843,.F.);
#87106=ORIENTED_EDGE('',*,*,#58837,.F.);
#87107=ORIENTED_EDGE('',*,*,#58819,.T.);
#87108=ORIENTED_EDGE('',*,*,#58824,.T.);
#87109=ORIENTED_EDGE('',*,*,#58812,.T.);
#87110=ORIENTED_EDGE('',*,*,#58808,.T.);
#87111=ORIENTED_EDGE('',*,*,#58805,.T.);
#87112=ORIENTED_EDGE('',*,*,#58802,.T.);
#87113=ORIENTED_EDGE('',*,*,#58799,.T.);
#87114=ORIENTED_EDGE('',*,*,#58796,.T.);
#87115=ORIENTED_EDGE('',*,*,#58793,.T.);
#87116=ORIENTED_EDGE('',*,*,#58815,.T.);
#87117=ORIENTED_EDGE('',*,*,#58849,.T.);
#87118=ORIENTED_EDGE('',*,*,#58786,.T.);
#87119=ORIENTED_EDGE('',*,*,#58783,.T.);
#87120=ORIENTED_EDGE('',*,*,#58780,.T.);
#87121=ORIENTED_EDGE('',*,*,#58777,.T.);
#87122=ORIENTED_EDGE('',*,*,#58774,.T.);
#87123=ORIENTED_EDGE('',*,*,#58771,.T.);
#87124=ORIENTED_EDGE('',*,*,#58784,.T.);
#87125=ORIENTED_EDGE('',*,*,#58849,.F.);
#87126=ORIENTED_EDGE('',*,*,#58814,.T.);
#87127=ORIENTED_EDGE('',*,*,#58850,.T.);
#87128=ORIENTED_EDGE('',*,*,#58820,.T.);
#87129=ORIENTED_EDGE('',*,*,#58769,.F.);
#87130=ORIENTED_EDGE('',*,*,#58773,.F.);
#87131=ORIENTED_EDGE('',*,*,#58776,.F.);
#87132=ORIENTED_EDGE('',*,*,#58779,.F.);
#87133=ORIENTED_EDGE('',*,*,#58782,.F.);
#87134=ORIENTED_EDGE('',*,*,#58785,.F.);
#87135=ORIENTED_EDGE('',*,*,#58850,.F.);
#87136=ORIENTED_EDGE('',*,*,#58813,.T.);
#87137=ORIENTED_EDGE('',*,*,#58788,.T.);
#87138=ORIENTED_EDGE('',*,*,#58791,.T.);
#87139=ORIENTED_EDGE('',*,*,#58795,.T.);
#87140=ORIENTED_EDGE('',*,*,#58798,.T.);
#87141=ORIENTED_EDGE('',*,*,#58801,.T.);
#87142=ORIENTED_EDGE('',*,*,#58804,.T.);
#87143=ORIENTED_EDGE('',*,*,#58807,.T.);
#87144=ORIENTED_EDGE('',*,*,#58811,.T.);
#87145=ORIENTED_EDGE('',*,*,#58851,.F.);
#87146=ORIENTED_EDGE('',*,*,#58852,.T.);
#87147=ORIENTED_EDGE('',*,*,#58853,.F.);
#87148=ORIENTED_EDGE('',*,*,#58852,.F.);
#87149=ORIENTED_EDGE('',*,*,#58854,.F.);
#87150=ORIENTED_EDGE('',*,*,#58855,.F.);
#87151=ORIENTED_EDGE('',*,*,#58856,.T.);
#87152=ORIENTED_EDGE('',*,*,#58857,.F.);
#87153=ORIENTED_EDGE('',*,*,#58856,.F.);
#87154=ORIENTED_EDGE('',*,*,#58858,.F.);
#87155=ORIENTED_EDGE('',*,*,#58859,.T.);
#87156=ORIENTED_EDGE('',*,*,#58860,.F.);
#87157=ORIENTED_EDGE('',*,*,#58859,.F.);
#87158=ORIENTED_EDGE('',*,*,#58861,.F.);
#87159=ORIENTED_EDGE('',*,*,#58862,.F.);
#87160=ORIENTED_EDGE('',*,*,#58863,.T.);
#87161=ORIENTED_EDGE('',*,*,#58864,.F.);
#87162=ORIENTED_EDGE('',*,*,#58863,.F.);
#87163=ORIENTED_EDGE('',*,*,#58861,.T.);
#87164=ORIENTED_EDGE('',*,*,#58862,.T.);
#87165=ORIENTED_EDGE('',*,*,#58865,.T.);
#87166=ORIENTED_EDGE('',*,*,#58866,.F.);
#87167=ORIENTED_EDGE('',*,*,#58867,.T.);
#87168=ORIENTED_EDGE('',*,*,#58858,.T.);
#87169=ORIENTED_EDGE('',*,*,#58867,.F.);
#87170=ORIENTED_EDGE('',*,*,#58868,.F.);
#87171=ORIENTED_EDGE('',*,*,#58865,.F.);
#87172=ORIENTED_EDGE('',*,*,#58869,.F.);
#87173=ORIENTED_EDGE('',*,*,#58870,.F.);
#87174=ORIENTED_EDGE('',*,*,#58869,.T.);
#87175=ORIENTED_EDGE('',*,*,#58871,.T.);
#87176=ORIENTED_EDGE('',*,*,#58872,.F.);
#87177=ORIENTED_EDGE('',*,*,#58871,.F.);
#87178=ORIENTED_EDGE('',*,*,#58870,.T.);
#87179=ORIENTED_EDGE('',*,*,#58866,.T.);
#87180=ORIENTED_EDGE('',*,*,#58868,.T.);
#87181=ORIENTED_EDGE('',*,*,#58873,.T.);
#87182=ORIENTED_EDGE('',*,*,#58874,.F.);
#87183=ORIENTED_EDGE('',*,*,#58875,.F.);
#87184=ORIENTED_EDGE('',*,*,#58873,.F.);
#87185=ORIENTED_EDGE('',*,*,#58854,.T.);
#87186=ORIENTED_EDGE('',*,*,#58855,.T.);
#87187=ORIENTED_EDGE('',*,*,#58876,.T.);
#87188=ORIENTED_EDGE('',*,*,#58875,.T.);
#87189=ORIENTED_EDGE('',*,*,#58877,.T.);
#87190=ORIENTED_EDGE('',*,*,#58851,.T.);
#87191=ORIENTED_EDGE('',*,*,#58877,.F.);
#87192=ORIENTED_EDGE('',*,*,#58874,.T.);
#87193=ORIENTED_EDGE('',*,*,#58876,.F.);
#87194=ORIENTED_EDGE('',*,*,#58872,.T.);
#87195=ORIENTED_EDGE('',*,*,#58860,.T.);
#87196=ORIENTED_EDGE('',*,*,#58857,.T.);
#87197=ORIENTED_EDGE('',*,*,#58864,.T.);
#87198=ORIENTED_EDGE('',*,*,#58853,.T.);
#87199=ORIENTED_EDGE('',*,*,#58878,.F.);
#87200=ORIENTED_EDGE('',*,*,#58879,.T.);
#87201=ORIENTED_EDGE('',*,*,#58880,.T.);
#87202=ORIENTED_EDGE('',*,*,#58879,.F.);
#87203=ORIENTED_EDGE('',*,*,#58881,.T.);
#87204=ORIENTED_EDGE('',*,*,#58882,.T.);
#87205=ORIENTED_EDGE('',*,*,#58883,.F.);
#87206=ORIENTED_EDGE('',*,*,#58882,.F.);
#87207=ORIENTED_EDGE('',*,*,#58884,.F.);
#87208=ORIENTED_EDGE('',*,*,#58885,.T.);
#87209=ORIENTED_EDGE('',*,*,#58886,.F.);
#87210=ORIENTED_EDGE('',*,*,#58887,.F.);
#87211=ORIENTED_EDGE('',*,*,#58885,.F.);
#87212=ORIENTED_EDGE('',*,*,#58888,.T.);
#87213=ORIENTED_EDGE('',*,*,#58889,.T.);
#87214=ORIENTED_EDGE('',*,*,#58886,.T.);
#87215=ORIENTED_EDGE('',*,*,#58887,.T.);
#87216=ORIENTED_EDGE('',*,*,#58889,.F.);
#87217=ORIENTED_EDGE('',*,*,#58890,.T.);
#87218=ORIENTED_EDGE('',*,*,#58891,.F.);
#87219=ORIENTED_EDGE('',*,*,#58892,.T.);
#87220=ORIENTED_EDGE('',*,*,#58893,.T.);
#87221=ORIENTED_EDGE('',*,*,#58894,.T.);
#87222=ORIENTED_EDGE('',*,*,#58895,.T.);
#87223=ORIENTED_EDGE('',*,*,#58896,.F.);
#87224=ORIENTED_EDGE('',*,*,#58895,.F.);
#87225=ORIENTED_EDGE('',*,*,#58897,.F.);
#87226=ORIENTED_EDGE('',*,*,#58898,.T.);
#87227=ORIENTED_EDGE('',*,*,#58899,.T.);
#87228=ORIENTED_EDGE('',*,*,#58898,.F.);
#87229=ORIENTED_EDGE('',*,*,#58900,.F.);
#87230=ORIENTED_EDGE('',*,*,#58901,.T.);
#87231=ORIENTED_EDGE('',*,*,#58902,.T.);
#87232=ORIENTED_EDGE('',*,*,#58901,.F.);
#87233=ORIENTED_EDGE('',*,*,#58903,.F.);
#87234=ORIENTED_EDGE('',*,*,#58904,.T.);
#87235=ORIENTED_EDGE('',*,*,#58905,.T.);
#87236=ORIENTED_EDGE('',*,*,#58904,.F.);
#87237=ORIENTED_EDGE('',*,*,#58906,.F.);
#87238=ORIENTED_EDGE('',*,*,#58907,.T.);
#87239=ORIENTED_EDGE('',*,*,#58908,.T.);
#87240=ORIENTED_EDGE('',*,*,#58907,.F.);
#87241=ORIENTED_EDGE('',*,*,#58909,.F.);
#87242=ORIENTED_EDGE('',*,*,#58910,.T.);
#87243=ORIENTED_EDGE('',*,*,#58911,.T.);
#87244=ORIENTED_EDGE('',*,*,#58910,.F.);
#87245=ORIENTED_EDGE('',*,*,#58912,.T.);
#87246=ORIENTED_EDGE('',*,*,#58913,.T.);
#87247=ORIENTED_EDGE('',*,*,#58914,.F.);
#87248=ORIENTED_EDGE('',*,*,#58913,.F.);
#87249=ORIENTED_EDGE('',*,*,#58915,.T.);
#87250=ORIENTED_EDGE('',*,*,#58916,.T.);
#87251=ORIENTED_EDGE('',*,*,#58917,.F.);
#87252=ORIENTED_EDGE('',*,*,#58916,.F.);
#87253=ORIENTED_EDGE('',*,*,#58918,.T.);
#87254=ORIENTED_EDGE('',*,*,#58919,.T.);
#87255=ORIENTED_EDGE('',*,*,#58920,.F.);
#87256=ORIENTED_EDGE('',*,*,#58919,.F.);
#87257=ORIENTED_EDGE('',*,*,#58921,.T.);
#87258=ORIENTED_EDGE('',*,*,#58922,.T.);
#87259=ORIENTED_EDGE('',*,*,#58923,.F.);
#87260=ORIENTED_EDGE('',*,*,#58922,.F.);
#87261=ORIENTED_EDGE('',*,*,#58924,.T.);
#87262=ORIENTED_EDGE('',*,*,#58925,.T.);
#87263=ORIENTED_EDGE('',*,*,#58926,.F.);
#87264=ORIENTED_EDGE('',*,*,#58927,.F.);
#87265=ORIENTED_EDGE('',*,*,#58926,.T.);
#87266=ORIENTED_EDGE('',*,*,#58928,.T.);
#87267=ORIENTED_EDGE('',*,*,#58929,.F.);
#87268=ORIENTED_EDGE('',*,*,#58930,.F.);
#87269=ORIENTED_EDGE('',*,*,#58929,.T.);
#87270=ORIENTED_EDGE('',*,*,#58931,.T.);
#87271=ORIENTED_EDGE('',*,*,#58932,.F.);
#87272=ORIENTED_EDGE('',*,*,#58933,.F.);
#87273=ORIENTED_EDGE('',*,*,#58932,.T.);
#87274=ORIENTED_EDGE('',*,*,#58934,.T.);
#87275=ORIENTED_EDGE('',*,*,#58935,.F.);
#87276=ORIENTED_EDGE('',*,*,#58936,.F.);
#87277=ORIENTED_EDGE('',*,*,#58935,.T.);
#87278=ORIENTED_EDGE('',*,*,#58937,.T.);
#87279=ORIENTED_EDGE('',*,*,#58938,.F.);
#87280=ORIENTED_EDGE('',*,*,#58939,.F.);
#87281=ORIENTED_EDGE('',*,*,#58938,.T.);
#87282=ORIENTED_EDGE('',*,*,#58940,.T.);
#87283=ORIENTED_EDGE('',*,*,#58941,.F.);
#87284=ORIENTED_EDGE('',*,*,#58942,.F.);
#87285=ORIENTED_EDGE('',*,*,#58941,.T.);
#87286=ORIENTED_EDGE('',*,*,#58943,.T.);
#87287=ORIENTED_EDGE('',*,*,#58944,.F.);
#87288=ORIENTED_EDGE('',*,*,#58945,.F.);
#87289=ORIENTED_EDGE('',*,*,#58944,.T.);
#87290=ORIENTED_EDGE('',*,*,#58946,.T.);
#87291=ORIENTED_EDGE('',*,*,#58924,.F.);
#87292=ORIENTED_EDGE('',*,*,#58947,.F.);
#87293=ORIENTED_EDGE('',*,*,#58948,.T.);
#87294=ORIENTED_EDGE('',*,*,#58949,.T.);
#87295=ORIENTED_EDGE('',*,*,#58950,.T.);
#87296=ORIENTED_EDGE('',*,*,#58951,.T.);
#87297=ORIENTED_EDGE('',*,*,#58952,.T.);
#87298=ORIENTED_EDGE('',*,*,#58953,.T.);
#87299=ORIENTED_EDGE('',*,*,#58954,.T.);
#87300=ORIENTED_EDGE('',*,*,#58955,.T.);
#87301=ORIENTED_EDGE('',*,*,#58900,.T.);
#87302=ORIENTED_EDGE('',*,*,#58903,.T.);
#87303=ORIENTED_EDGE('',*,*,#58906,.T.);
#87304=ORIENTED_EDGE('',*,*,#58909,.T.);
#87305=ORIENTED_EDGE('',*,*,#58896,.T.);
#87306=ORIENTED_EDGE('',*,*,#58911,.F.);
#87307=ORIENTED_EDGE('',*,*,#58914,.T.);
#87308=ORIENTED_EDGE('',*,*,#58908,.F.);
#87309=ORIENTED_EDGE('',*,*,#58917,.T.);
#87310=ORIENTED_EDGE('',*,*,#58905,.F.);
#87311=ORIENTED_EDGE('',*,*,#58920,.T.);
#87312=ORIENTED_EDGE('',*,*,#58902,.F.);
#87313=ORIENTED_EDGE('',*,*,#58923,.T.);
#87314=ORIENTED_EDGE('',*,*,#58956,.F.);
#87315=ORIENTED_EDGE('',*,*,#58957,.F.);
#87316=ORIENTED_EDGE('',*,*,#58958,.F.);
#87317=ORIENTED_EDGE('',*,*,#58959,.F.);
#87318=ORIENTED_EDGE('',*,*,#58960,.F.);
#87319=ORIENTED_EDGE('',*,*,#58961,.F.);
#87320=ORIENTED_EDGE('',*,*,#58962,.F.);
#87321=ORIENTED_EDGE('',*,*,#58963,.F.);
#87322=ORIENTED_EDGE('',*,*,#58947,.T.);
#87323=ORIENTED_EDGE('',*,*,#58927,.T.);
#87324=ORIENTED_EDGE('',*,*,#58930,.T.);
#87325=ORIENTED_EDGE('',*,*,#58933,.T.);
#87326=ORIENTED_EDGE('',*,*,#58936,.T.);
#87327=ORIENTED_EDGE('',*,*,#58939,.T.);
#87328=ORIENTED_EDGE('',*,*,#58942,.T.);
#87329=ORIENTED_EDGE('',*,*,#58945,.T.);
#87330=ORIENTED_EDGE('',*,*,#58956,.T.);
#87331=ORIENTED_EDGE('',*,*,#58964,.F.);
#87332=ORIENTED_EDGE('',*,*,#58965,.F.);
#87333=ORIENTED_EDGE('',*,*,#58966,.T.);
#87334=ORIENTED_EDGE('',*,*,#58963,.T.);
#87335=ORIENTED_EDGE('',*,*,#58967,.F.);
#87336=ORIENTED_EDGE('',*,*,#58968,.F.);
#87337=ORIENTED_EDGE('',*,*,#58964,.T.);
#87338=ORIENTED_EDGE('',*,*,#58962,.T.);
#87339=ORIENTED_EDGE('',*,*,#58969,.F.);
#87340=ORIENTED_EDGE('',*,*,#58970,.F.);
#87341=ORIENTED_EDGE('',*,*,#58967,.T.);
#87342=ORIENTED_EDGE('',*,*,#58961,.T.);
#87343=ORIENTED_EDGE('',*,*,#58971,.F.);
#87344=ORIENTED_EDGE('',*,*,#58972,.F.);
#87345=ORIENTED_EDGE('',*,*,#58969,.T.);
#87346=ORIENTED_EDGE('',*,*,#58960,.T.);
#87347=ORIENTED_EDGE('',*,*,#58973,.F.);
#87348=ORIENTED_EDGE('',*,*,#58974,.F.);
#87349=ORIENTED_EDGE('',*,*,#58971,.T.);
#87350=ORIENTED_EDGE('',*,*,#58959,.T.);
#87351=ORIENTED_EDGE('',*,*,#58975,.F.);
#87352=ORIENTED_EDGE('',*,*,#58976,.F.);
#87353=ORIENTED_EDGE('',*,*,#58973,.T.);
#87354=ORIENTED_EDGE('',*,*,#58958,.T.);
#87355=ORIENTED_EDGE('',*,*,#58977,.F.);
#87356=ORIENTED_EDGE('',*,*,#58978,.F.);
#87357=ORIENTED_EDGE('',*,*,#58975,.T.);
#87358=ORIENTED_EDGE('',*,*,#58957,.T.);
#87359=ORIENTED_EDGE('',*,*,#58966,.F.);
#87360=ORIENTED_EDGE('',*,*,#58979,.F.);
#87361=ORIENTED_EDGE('',*,*,#58977,.T.);
#87362=ORIENTED_EDGE('',*,*,#58980,.F.);
#87363=ORIENTED_EDGE('',*,*,#58953,.F.);
#87364=ORIENTED_EDGE('',*,*,#58981,.F.);
#87365=ORIENTED_EDGE('',*,*,#58937,.F.);
#87366=ORIENTED_EDGE('',*,*,#58981,.T.);
#87367=ORIENTED_EDGE('',*,*,#58952,.F.);
#87368=ORIENTED_EDGE('',*,*,#58982,.F.);
#87369=ORIENTED_EDGE('',*,*,#58940,.F.);
#87370=ORIENTED_EDGE('',*,*,#58980,.T.);
#87371=ORIENTED_EDGE('',*,*,#58934,.F.);
#87372=ORIENTED_EDGE('',*,*,#58983,.F.);
#87373=ORIENTED_EDGE('',*,*,#58954,.F.);
#87374=ORIENTED_EDGE('',*,*,#58982,.T.);
#87375=ORIENTED_EDGE('',*,*,#58951,.F.);
#87376=ORIENTED_EDGE('',*,*,#58984,.F.);
#87377=ORIENTED_EDGE('',*,*,#58943,.F.);
#87378=ORIENTED_EDGE('',*,*,#58983,.T.);
#87379=ORIENTED_EDGE('',*,*,#58931,.F.);
#87380=ORIENTED_EDGE('',*,*,#58985,.F.);
#87381=ORIENTED_EDGE('',*,*,#58955,.F.);
#87382=ORIENTED_EDGE('',*,*,#58984,.T.);
#87383=ORIENTED_EDGE('',*,*,#58950,.F.);
#87384=ORIENTED_EDGE('',*,*,#58986,.F.);
#87385=ORIENTED_EDGE('',*,*,#58946,.F.);
#87386=ORIENTED_EDGE('',*,*,#58985,.T.);
#87387=ORIENTED_EDGE('',*,*,#58928,.F.);
#87388=ORIENTED_EDGE('',*,*,#58987,.F.);
#87389=ORIENTED_EDGE('',*,*,#58948,.F.);
#87390=ORIENTED_EDGE('',*,*,#58986,.T.);
#87391=ORIENTED_EDGE('',*,*,#58949,.F.);
#87392=ORIENTED_EDGE('',*,*,#58987,.T.);
#87393=ORIENTED_EDGE('',*,*,#58925,.F.);
#87394=ORIENTED_EDGE('',*,*,#58965,.T.);
#87395=ORIENTED_EDGE('',*,*,#58968,.T.);
#87396=ORIENTED_EDGE('',*,*,#58970,.T.);
#87397=ORIENTED_EDGE('',*,*,#58972,.T.);
#87398=ORIENTED_EDGE('',*,*,#58974,.T.);
#87399=ORIENTED_EDGE('',*,*,#58976,.T.);
#87400=ORIENTED_EDGE('',*,*,#58978,.T.);
#87401=ORIENTED_EDGE('',*,*,#58979,.T.);
#87402=ORIENTED_EDGE('',*,*,#58912,.F.);
#87403=ORIENTED_EDGE('',*,*,#58918,.F.);
#87404=ORIENTED_EDGE('',*,*,#58899,.F.);
#87405=ORIENTED_EDGE('',*,*,#58915,.F.);
#87406=ORIENTED_EDGE('',*,*,#58921,.F.);
#87407=ORIENTED_EDGE('',*,*,#58988,.T.);
#87408=ORIENTED_EDGE('',*,*,#58989,.T.);
#87409=ORIENTED_EDGE('',*,*,#58990,.F.);
#87410=ORIENTED_EDGE('',*,*,#58991,.T.);
#87411=ORIENTED_EDGE('',*,*,#58884,.T.);
#87412=ORIENTED_EDGE('',*,*,#58992,.T.);
#87413=ORIENTED_EDGE('',*,*,#58993,.T.);
#87414=ORIENTED_EDGE('',*,*,#58994,.T.);
#87415=ORIENTED_EDGE('',*,*,#58890,.F.);
#87416=ORIENTED_EDGE('',*,*,#58995,.F.);
#87417=ORIENTED_EDGE('',*,*,#58996,.F.);
#87418=ORIENTED_EDGE('',*,*,#58997,.F.);
#87419=ORIENTED_EDGE('',*,*,#58989,.F.);
#87420=ORIENTED_EDGE('',*,*,#58894,.F.);
#87421=ORIENTED_EDGE('',*,*,#58883,.T.);
#87422=ORIENTED_EDGE('',*,*,#58897,.T.);
#87423=ORIENTED_EDGE('',*,*,#58888,.F.);
#87424=ORIENTED_EDGE('',*,*,#58878,.T.);
#87425=ORIENTED_EDGE('',*,*,#58881,.F.);
#87426=ORIENTED_EDGE('',*,*,#58996,.T.);
#87427=ORIENTED_EDGE('',*,*,#58998,.F.);
#87428=ORIENTED_EDGE('',*,*,#58999,.F.);
#87429=ORIENTED_EDGE('',*,*,#59000,.T.);
#87430=ORIENTED_EDGE('',*,*,#58997,.T.);
#87431=ORIENTED_EDGE('',*,*,#59000,.F.);
#87432=ORIENTED_EDGE('',*,*,#59001,.F.);
#87433=ORIENTED_EDGE('',*,*,#58990,.T.);
#87434=ORIENTED_EDGE('',*,*,#58995,.T.);
#87435=ORIENTED_EDGE('',*,*,#58893,.F.);
#87436=ORIENTED_EDGE('',*,*,#59002,.F.);
#87437=ORIENTED_EDGE('',*,*,#58998,.T.);
#87438=ORIENTED_EDGE('',*,*,#58999,.T.);
#87439=ORIENTED_EDGE('',*,*,#59002,.T.);
#87440=ORIENTED_EDGE('',*,*,#58892,.F.);
#87441=ORIENTED_EDGE('',*,*,#59003,.F.);
#87442=ORIENTED_EDGE('',*,*,#59004,.F.);
#87443=ORIENTED_EDGE('',*,*,#59005,.F.);
#87444=ORIENTED_EDGE('',*,*,#58991,.F.);
#87445=ORIENTED_EDGE('',*,*,#59001,.T.);
#87446=ORIENTED_EDGE('',*,*,#58880,.F.);
#87447=ORIENTED_EDGE('',*,*,#58993,.F.);
#87448=ORIENTED_EDGE('',*,*,#59006,.F.);
#87449=ORIENTED_EDGE('',*,*,#59004,.T.);
#87450=ORIENTED_EDGE('',*,*,#59007,.T.);
#87451=ORIENTED_EDGE('',*,*,#58992,.F.);
#87452=ORIENTED_EDGE('',*,*,#58988,.F.);
#87453=ORIENTED_EDGE('',*,*,#59005,.T.);
#87454=ORIENTED_EDGE('',*,*,#59006,.T.);
#87455=ORIENTED_EDGE('',*,*,#58994,.F.);
#87456=ORIENTED_EDGE('',*,*,#59007,.F.);
#87457=ORIENTED_EDGE('',*,*,#59003,.T.);
#87458=ORIENTED_EDGE('',*,*,#58891,.T.);
#90343=CYLINDRICAL_SURFACE('',#98945,0.508000000000002);
#90344=CYLINDRICAL_SURFACE('',#98948,5.1435);
#90345=CYLINDRICAL_SURFACE('',#98972,0.952499999999998);
#90346=CYLINDRICAL_SURFACE('',#99000,0.508000000000002);
#90347=CYLINDRICAL_SURFACE('',#99001,0.508000000000002);
#90348=CYLINDRICAL_SURFACE('',#99002,0.508000000000002);
#90349=CYLINDRICAL_SURFACE('',#99003,0.508000000000002);
#90350=CYLINDRICAL_SURFACE('',#99004,0.508000000000002);
#90351=CYLINDRICAL_SURFACE('',#99005,7.9375);
#90352=CYLINDRICAL_SURFACE('',#99008,8.4455);
#90353=CYLINDRICAL_SURFACE('',#99013,7.9375);
#90354=CYLINDRICAL_SURFACE('',#99016,8.4455);
#90355=CYLINDRICAL_SURFACE('',#99021,7.9375);
#90356=CYLINDRICAL_SURFACE('',#99024,8.4455);
#90357=CYLINDRICAL_SURFACE('',#99029,7.9375);
#90358=CYLINDRICAL_SURFACE('',#99032,8.4455);
#90359=CYLINDRICAL_SURFACE('',#99047,51.27);
#90360=CYLINDRICAL_SURFACE('',#99049,50.);
#90361=CYLINDRICAL_SURFACE('',#99063,56.875);
#90362=CYLINDRICAL_SURFACE('',#99065,55.605);
#90363=CYLINDRICAL_SURFACE('',#99069,51.27);
#90364=CYLINDRICAL_SURFACE('',#99072,55.605);
#90365=CYLINDRICAL_SURFACE('',#99116,65.);
#90366=CYLINDRICAL_SURFACE('',#99362,56.875);
#90367=CYLINDRICAL_SURFACE('',#101120,0.175259999999997);
#90368=CYLINDRICAL_SURFACE('',#101121,0.175259999999997);
#90369=CYLINDRICAL_SURFACE('',#101122,0.126999999706107);
#90370=CYLINDRICAL_SURFACE('',#101126,0.127000000000002);
#90371=CYLINDRICAL_SURFACE('',#101128,0.127000000000002);
#90372=CYLINDRICAL_SURFACE('',#101132,0.127000005437004);
#90373=CYLINDRICAL_SURFACE('',#101134,0.12700000128033);
#90374=CYLINDRICAL_SURFACE('',#101137,0.127000000000002);
#90375=CYLINDRICAL_SURFACE('',#101143,0.126999993615305);
#90376=CYLINDRICAL_SURFACE('',#101145,0.127000005453425);
#90377=CYLINDRICAL_SURFACE('',#101151,0.127000000000002);
#90378=CYLINDRICAL_SURFACE('',#101154,0.126999998754292);
#90379=CYLINDRICAL_SURFACE('',#101156,0.126999993594532);
#90380=CYLINDRICAL_SURFACE('',#101160,0.127000000000002);
#90381=CYLINDRICAL_SURFACE('',#101162,0.127000000000002);
#90382=CYLINDRICAL_SURFACE('',#101165,0.127000000300332);
#90383=CYLINDRICAL_SURFACE('',#101929,0.175259999999999);
#90384=CYLINDRICAL_SURFACE('',#101930,0.17526);
#90385=CYLINDRICAL_SURFACE('',#101931,0.175259999999999);
#90386=CYLINDRICAL_SURFACE('',#101932,0.17526);
#90387=CYLINDRICAL_SURFACE('',#101933,0.175259999999999);
#90388=CYLINDRICAL_SURFACE('',#101934,0.17526);
#90389=CYLINDRICAL_SURFACE('',#101935,0.17526);
#90390=CYLINDRICAL_SURFACE('',#101936,0.17526);
#90391=CYLINDRICAL_SURFACE('',#101937,0.175259999999998);
#90392=CYLINDRICAL_SURFACE('',#101938,0.17526);
#90393=CYLINDRICAL_SURFACE('',#101939,0.17526);
#90394=CYLINDRICAL_SURFACE('',#101940,0.17526);
#90395=CYLINDRICAL_SURFACE('',#101941,0.175260000000001);
#90396=CYLINDRICAL_SURFACE('',#101942,0.17526);
#90397=CYLINDRICAL_SURFACE('',#101943,0.175260000000001);
#90398=CYLINDRICAL_SURFACE('',#101944,0.17526);
#90399=CYLINDRICAL_SURFACE('',#101945,0.17526);
#90400=CYLINDRICAL_SURFACE('',#101946,0.17526);
#90401=CYLINDRICAL_SURFACE('',#101947,0.175260000000001);
#90402=CYLINDRICAL_SURFACE('',#101948,0.17526);
#90403=CYLINDRICAL_SURFACE('',#101949,0.17526);
#90404=CYLINDRICAL_SURFACE('',#101950,0.17526);
#90405=CYLINDRICAL_SURFACE('',#101951,0.175259999999999);
#90406=CYLINDRICAL_SURFACE('',#101952,0.17526);
#90407=CYLINDRICAL_SURFACE('',#101953,0.175259999999999);
#90408=CYLINDRICAL_SURFACE('',#101954,0.17526);
#90409=CYLINDRICAL_SURFACE('',#101955,0.175259999999999);
#90410=CYLINDRICAL_SURFACE('',#101956,0.17526);
#90411=CYLINDRICAL_SURFACE('',#101957,0.17526);
#90412=CYLINDRICAL_SURFACE('',#101958,0.17526);
#90413=CYLINDRICAL_SURFACE('',#101959,0.175259999999999);
#90414=CYLINDRICAL_SURFACE('',#101960,0.17526);
#90415=CYLINDRICAL_SURFACE('',#101961,0.17526);
#90416=CYLINDRICAL_SURFACE('',#101962,0.17526);
#90417=CYLINDRICAL_SURFACE('',#101963,0.175259999999999);
#90418=CYLINDRICAL_SURFACE('',#101964,0.17526);
#90419=CYLINDRICAL_SURFACE('',#101965,0.17526);
#90420=CYLINDRICAL_SURFACE('',#101966,0.17526);
#90421=CYLINDRICAL_SURFACE('',#101967,0.175259999999998);
#90422=CYLINDRICAL_SURFACE('',#101968,0.17526);
#90423=CYLINDRICAL_SURFACE('',#101969,0.17526);
#90424=CYLINDRICAL_SURFACE('',#101970,0.17526);
#90425=CYLINDRICAL_SURFACE('',#101971,0.175260000000001);
#90426=CYLINDRICAL_SURFACE('',#101972,0.17526);
#90427=CYLINDRICAL_SURFACE('',#101973,0.175260000000001);
#90428=CYLINDRICAL_SURFACE('',#101974,0.17526);
#90429=CYLINDRICAL_SURFACE('',#101975,0.17526);
#90430=CYLINDRICAL_SURFACE('',#101976,0.17526);
#90431=CYLINDRICAL_SURFACE('',#101977,0.175260000000001);
#90432=CYLINDRICAL_SURFACE('',#101978,0.17526);
#90433=CYLINDRICAL_SURFACE('',#101979,0.175260000000003);
#90434=CYLINDRICAL_SURFACE('',#101980,0.17526);
#90435=CYLINDRICAL_SURFACE('',#101981,0.175259999999999);
#90436=CYLINDRICAL_SURFACE('',#101982,0.17526);
#90437=CYLINDRICAL_SURFACE('',#101983,0.175259999999999);
#90438=CYLINDRICAL_SURFACE('',#101984,0.17526);
#90439=CYLINDRICAL_SURFACE('',#101985,0.17526);
#90440=CYLINDRICAL_SURFACE('',#101986,0.17526);
#90441=CYLINDRICAL_SURFACE('',#101987,0.175259999999997);
#90442=CYLINDRICAL_SURFACE('',#101988,0.175259999999997);
#90443=CYLINDRICAL_SURFACE('',#101989,0.17526);
#90444=CYLINDRICAL_SURFACE('',#101990,0.17526);
#90445=CYLINDRICAL_SURFACE('',#101991,0.17526);
#90446=CYLINDRICAL_SURFACE('',#101992,0.17526);
#90447=CYLINDRICAL_SURFACE('',#101993,0.175259999999999);
#90448=CYLINDRICAL_SURFACE('',#101994,0.17526);
#90449=CYLINDRICAL_SURFACE('',#101995,0.17526);
#90450=CYLINDRICAL_SURFACE('',#101996,0.17526);
#90451=CYLINDRICAL_SURFACE('',#101997,0.175259999999998);
#90452=CYLINDRICAL_SURFACE('',#101998,0.17526);
#90453=CYLINDRICAL_SURFACE('',#101999,0.17526);
#90454=CYLINDRICAL_SURFACE('',#102000,0.17526);
#90455=CYLINDRICAL_SURFACE('',#102001,0.175259999999996);
#90456=CYLINDRICAL_SURFACE('',#102002,0.17526);
#90457=CYLINDRICAL_SURFACE('',#102003,0.175260000000001);
#90458=CYLINDRICAL_SURFACE('',#102004,0.17526);
#90459=CYLINDRICAL_SURFACE('',#102005,0.175259999999995);
#90460=CYLINDRICAL_SURFACE('',#102006,0.17526);
#90461=CYLINDRICAL_SURFACE('',#102007,0.175260000000001);
#90462=CYLINDRICAL_SURFACE('',#102008,0.17526);
#90463=CYLINDRICAL_SURFACE('',#102009,0.17526);
#90464=CYLINDRICAL_SURFACE('',#102010,0.17526);
#90465=CYLINDRICAL_SURFACE('',#102011,0.175259999999999);
#90466=CYLINDRICAL_SURFACE('',#102012,0.17526);
#90467=CYLINDRICAL_SURFACE('',#102013,0.175259999999999);
#90468=CYLINDRICAL_SURFACE('',#102014,0.17526);
#90469=CYLINDRICAL_SURFACE('',#102015,0.17526);
#90470=CYLINDRICAL_SURFACE('',#102016,0.17526);
#90471=CYLINDRICAL_SURFACE('',#102017,0.17526);
#90472=CYLINDRICAL_SURFACE('',#102018,0.17526);
#90473=CYLINDRICAL_SURFACE('',#102019,0.17526);
#90474=CYLINDRICAL_SURFACE('',#102020,0.17526);
#90475=CYLINDRICAL_SURFACE('',#102021,0.17526);
#90476=CYLINDRICAL_SURFACE('',#102022,0.17526);
#90477=CYLINDRICAL_SURFACE('',#102023,0.175259999999999);
#90478=CYLINDRICAL_SURFACE('',#102024,0.17526);
#90479=CYLINDRICAL_SURFACE('',#102025,0.17526);
#90480=CYLINDRICAL_SURFACE('',#102026,0.17526);
#90481=CYLINDRICAL_SURFACE('',#102027,0.175260000000001);
#90482=CYLINDRICAL_SURFACE('',#102028,0.17526);
#90483=CYLINDRICAL_SURFACE('',#102029,0.17526);
#90484=CYLINDRICAL_SURFACE('',#102030,0.17526);
#90485=CYLINDRICAL_SURFACE('',#102031,0.175259999999996);
#90486=CYLINDRICAL_SURFACE('',#102032,0.17526);
#90487=CYLINDRICAL_SURFACE('',#102033,0.175260000000001);
#90488=CYLINDRICAL_SURFACE('',#102034,0.17526);
#90489=CYLINDRICAL_SURFACE('',#102035,0.175260000000001);
#90490=CYLINDRICAL_SURFACE('',#102036,0.17526);
#90491=CYLINDRICAL_SURFACE('',#102037,0.175260000000001);
#90492=CYLINDRICAL_SURFACE('',#102038,0.17526);
#90493=CYLINDRICAL_SURFACE('',#102039,0.17526);
#90494=CYLINDRICAL_SURFACE('',#102040,0.17526);
#90495=CYLINDRICAL_SURFACE('',#102041,0.175259999999999);
#90496=CYLINDRICAL_SURFACE('',#102042,0.17526);
#90497=CYLINDRICAL_SURFACE('',#102043,0.175260000000001);
#90498=CYLINDRICAL_SURFACE('',#102044,0.17526);
#90499=CYLINDRICAL_SURFACE('',#102045,0.17526);
#90500=CYLINDRICAL_SURFACE('',#102046,0.17526);
#90501=CYLINDRICAL_SURFACE('',#102047,0.12699999970626);
#90502=CYLINDRICAL_SURFACE('',#102051,0.127);
#90503=CYLINDRICAL_SURFACE('',#102053,0.127);
#90504=CYLINDRICAL_SURFACE('',#102057,0.12700000543866);
#90505=CYLINDRICAL_SURFACE('',#102059,0.127000001278441);
#90506=CYLINDRICAL_SURFACE('',#102062,0.127);
#90507=CYLINDRICAL_SURFACE('',#102068,0.126999993613266);
#90508=CYLINDRICAL_SURFACE('',#102070,0.12700000545647);
#90509=CYLINDRICAL_SURFACE('',#102076,0.126999999999999);
#90510=CYLINDRICAL_SURFACE('',#102079,0.126999998753988);
#90511=CYLINDRICAL_SURFACE('',#102081,0.126999993594684);
#90512=CYLINDRICAL_SURFACE('',#102085,0.126999999999999);
#90513=CYLINDRICAL_SURFACE('',#102087,0.126999999999999);
#90514=CYLINDRICAL_SURFACE('',#102090,0.127000000302185);
#90515=CYLINDRICAL_SURFACE('',#102091,0.126999999706651);
#90516=CYLINDRICAL_SURFACE('',#102095,0.127);
#90517=CYLINDRICAL_SURFACE('',#102097,0.127);
#90518=CYLINDRICAL_SURFACE('',#102101,0.127000005437342);
#90519=CYLINDRICAL_SURFACE('',#102103,0.127000001278921);
#90520=CYLINDRICAL_SURFACE('',#102106,0.127);
#90521=CYLINDRICAL_SURFACE('',#102112,0.126999993613615);
#90522=CYLINDRICAL_SURFACE('',#102114,0.127000005453428);
#90523=CYLINDRICAL_SURFACE('',#102120,0.126999999999999);
#90524=CYLINDRICAL_SURFACE('',#102123,0.126999998753426);
#90525=CYLINDRICAL_SURFACE('',#102125,0.126999993596104);
#90526=CYLINDRICAL_SURFACE('',#102129,0.126999999999999);
#90527=CYLINDRICAL_SURFACE('',#102131,0.126999999999999);
#90528=CYLINDRICAL_SURFACE('',#102134,0.127000000302599);
#90529=CYLINDRICAL_SURFACE('',#102135,0.126999999706856);
#90530=CYLINDRICAL_SURFACE('',#102139,0.127);
#90531=CYLINDRICAL_SURFACE('',#102141,0.127);
#90532=CYLINDRICAL_SURFACE('',#102145,0.127000005440703);
#90533=CYLINDRICAL_SURFACE('',#102147,0.127000001279188);
#90534=CYLINDRICAL_SURFACE('',#102150,0.127);
#90535=CYLINDRICAL_SURFACE('',#102156,0.126999993614716);
#90536=CYLINDRICAL_SURFACE('',#102158,0.127000005454496);
#90537=CYLINDRICAL_SURFACE('',#102164,0.127000000000002);
#90538=CYLINDRICAL_SURFACE('',#102167,0.126999998752722);
#90539=CYLINDRICAL_SURFACE('',#102169,0.126999993594443);
#90540=CYLINDRICAL_SURFACE('',#102173,0.127000000000002);
#90541=CYLINDRICAL_SURFACE('',#102175,0.127000000000002);
#90542=CYLINDRICAL_SURFACE('',#102178,0.127000000302178);
#90543=CYLINDRICAL_SURFACE('',#102179,0.126999999705935);
#90544=CYLINDRICAL_SURFACE('',#102183,0.127);
#90545=CYLINDRICAL_SURFACE('',#102185,0.127);
#90546=CYLINDRICAL_SURFACE('',#102189,0.127000005438044);
#90547=CYLINDRICAL_SURFACE('',#102191,0.127000001278499);
#90548=CYLINDRICAL_SURFACE('',#102194,0.127);
#90549=CYLINDRICAL_SURFACE('',#102200,0.12699999361266);
#90550=CYLINDRICAL_SURFACE('',#102202,0.12700000545514);
#90551=CYLINDRICAL_SURFACE('',#102208,0.127000000000001);
#90552=CYLINDRICAL_SURFACE('',#102211,0.12699999875473);
#90553=CYLINDRICAL_SURFACE('',#102213,0.126999993593948);
#90554=CYLINDRICAL_SURFACE('',#102217,0.127000000000001);
#90555=CYLINDRICAL_SURFACE('',#102219,0.127000000000001);
#90556=CYLINDRICAL_SURFACE('',#102222,0.127000000303238);
#90557=CYLINDRICAL_SURFACE('',#102223,0.126999999706812);
#90558=CYLINDRICAL_SURFACE('',#102227,0.127);
#90559=CYLINDRICAL_SURFACE('',#102229,0.127);
#90560=CYLINDRICAL_SURFACE('',#102233,0.127000005438477);
#90561=CYLINDRICAL_SURFACE('',#102235,0.127000001279166);
#90562=CYLINDRICAL_SURFACE('',#102238,0.127);
#90563=CYLINDRICAL_SURFACE('',#102244,0.126999993615516);
#90564=CYLINDRICAL_SURFACE('',#102246,0.127000005451529);
#90565=CYLINDRICAL_SURFACE('',#102252,0.127);
#90566=CYLINDRICAL_SURFACE('',#102255,0.126999998753742);
#90567=CYLINDRICAL_SURFACE('',#102257,0.126999993594221);
#90568=CYLINDRICAL_SURFACE('',#102261,0.127);
#90569=CYLINDRICAL_SURFACE('',#102263,0.127);
#90570=CYLINDRICAL_SURFACE('',#102266,0.127000000301966);
#90571=CYLINDRICAL_SURFACE('',#102267,0.126999999706062);
#90572=CYLINDRICAL_SURFACE('',#102271,0.127);
#90573=CYLINDRICAL_SURFACE('',#102273,0.127);
#90574=CYLINDRICAL_SURFACE('',#102277,0.127000005437502);
#90575=CYLINDRICAL_SURFACE('',#102279,0.127000001278692);
#90576=CYLINDRICAL_SURFACE('',#102282,0.127);
#90577=CYLINDRICAL_SURFACE('',#102288,0.126999993615408);
#90578=CYLINDRICAL_SURFACE('',#102290,0.127000005455299);
#90579=CYLINDRICAL_SURFACE('',#102296,0.127000000000001);
#90580=CYLINDRICAL_SURFACE('',#102299,0.126999998754172);
#90581=CYLINDRICAL_SURFACE('',#102301,0.126999993593136);
#90582=CYLINDRICAL_SURFACE('',#102305,0.127000000000001);
#90583=CYLINDRICAL_SURFACE('',#102307,0.127000000000001);
#90584=CYLINDRICAL_SURFACE('',#102310,0.127000000300007);
#90585=CYLINDRICAL_SURFACE('',#102311,0.126999999707742);
#90586=CYLINDRICAL_SURFACE('',#102315,0.127);
#90587=CYLINDRICAL_SURFACE('',#102317,0.127);
#90588=CYLINDRICAL_SURFACE('',#102321,0.127000005438627);
#90589=CYLINDRICAL_SURFACE('',#102323,0.127000001278838);
#90590=CYLINDRICAL_SURFACE('',#102326,0.127);
#90591=CYLINDRICAL_SURFACE('',#102332,0.126999993616684);
#90592=CYLINDRICAL_SURFACE('',#102334,0.127000005454564);
#90593=CYLINDRICAL_SURFACE('',#102340,0.126999999999998);
#90594=CYLINDRICAL_SURFACE('',#102343,0.126999998752247);
#90595=CYLINDRICAL_SURFACE('',#102345,0.126999993594708);
#90596=CYLINDRICAL_SURFACE('',#102349,0.126999999999998);
#90597=CYLINDRICAL_SURFACE('',#102351,0.126999999999998);
#90598=CYLINDRICAL_SURFACE('',#102354,0.127000000303882);
#90599=CYLINDRICAL_SURFACE('',#102355,0.126999999707639);
#90600=CYLINDRICAL_SURFACE('',#102359,0.127);
#90601=CYLINDRICAL_SURFACE('',#102361,0.127);
#90602=CYLINDRICAL_SURFACE('',#102365,0.127000005438079);
#90603=CYLINDRICAL_SURFACE('',#102367,0.127000001278142);
#90604=CYLINDRICAL_SURFACE('',#102370,0.127);
#90605=CYLINDRICAL_SURFACE('',#102376,0.126999993613654);
#90606=CYLINDRICAL_SURFACE('',#102378,0.127000005454222);
#90607=CYLINDRICAL_SURFACE('',#102384,0.127);
#90608=CYLINDRICAL_SURFACE('',#102387,0.126999998752798);
#90609=CYLINDRICAL_SURFACE('',#102389,0.126999993596256);
#90610=CYLINDRICAL_SURFACE('',#102393,0.127);
#90611=CYLINDRICAL_SURFACE('',#102395,0.127);
#90612=CYLINDRICAL_SURFACE('',#102398,0.127000000302042);
#90613=CYLINDRICAL_SURFACE('',#102399,0.126999999706423);
#90614=CYLINDRICAL_SURFACE('',#102403,0.127);
#90615=CYLINDRICAL_SURFACE('',#102405,0.127);
#90616=CYLINDRICAL_SURFACE('',#102409,0.127000005437262);
#90617=CYLINDRICAL_SURFACE('',#102411,0.127000001279889);
#90618=CYLINDRICAL_SURFACE('',#102414,0.127);
#90619=CYLINDRICAL_SURFACE('',#102420,0.126999993614019);
#90620=CYLINDRICAL_SURFACE('',#102422,0.127000005452903);
#90621=CYLINDRICAL_SURFACE('',#102428,0.126999999999999);
#90622=CYLINDRICAL_SURFACE('',#102431,0.126999998754081);
#90623=CYLINDRICAL_SURFACE('',#102433,0.126999993593342);
#90624=CYLINDRICAL_SURFACE('',#102437,0.126999999999999);
#90625=CYLINDRICAL_SURFACE('',#102439,0.126999999999999);
#90626=CYLINDRICAL_SURFACE('',#102442,0.127000000301453);
#90627=CYLINDRICAL_SURFACE('',#102443,0.12699999970728);
#90628=CYLINDRICAL_SURFACE('',#102447,0.127);
#90629=CYLINDRICAL_SURFACE('',#102449,0.127);
#90630=CYLINDRICAL_SURFACE('',#102453,0.12700000543635);
#90631=CYLINDRICAL_SURFACE('',#102455,0.127000001280708);
#90632=CYLINDRICAL_SURFACE('',#102458,0.127);
#90633=CYLINDRICAL_SURFACE('',#102464,0.126999993613472);
#90634=CYLINDRICAL_SURFACE('',#102466,0.127000005453988);
#90635=CYLINDRICAL_SURFACE('',#102472,0.127);
#90636=CYLINDRICAL_SURFACE('',#102475,0.12699999875345);
#90637=CYLINDRICAL_SURFACE('',#102477,0.126999993596425);
#90638=CYLINDRICAL_SURFACE('',#102481,0.127000000000001);
#90639=CYLINDRICAL_SURFACE('',#102483,0.127000000000001);
#90640=CYLINDRICAL_SURFACE('',#102486,0.127000000302115);
#90641=CYLINDRICAL_SURFACE('',#102487,0.126999999706815);
#90642=CYLINDRICAL_SURFACE('',#102491,0.127);
#90643=CYLINDRICAL_SURFACE('',#102493,0.127);
#90644=CYLINDRICAL_SURFACE('',#102497,0.127000005436472);
#90645=CYLINDRICAL_SURFACE('',#102499,0.127000001280011);
#90646=CYLINDRICAL_SURFACE('',#102502,0.127);
#90647=CYLINDRICAL_SURFACE('',#102508,0.126999993613169);
#90648=CYLINDRICAL_SURFACE('',#102510,0.127000005455449);
#90649=CYLINDRICAL_SURFACE('',#102516,0.127000000000001);
#90650=CYLINDRICAL_SURFACE('',#102519,0.126999998752879);
#90651=CYLINDRICAL_SURFACE('',#102521,0.126999993596861);
#90652=CYLINDRICAL_SURFACE('',#102525,0.127000000000001);
#90653=CYLINDRICAL_SURFACE('',#102527,0.127000000000001);
#90654=CYLINDRICAL_SURFACE('',#102530,0.127000000301642);
#90655=CYLINDRICAL_SURFACE('',#102531,0.126999999706798);
#90656=CYLINDRICAL_SURFACE('',#102535,0.127);
#90657=CYLINDRICAL_SURFACE('',#102537,0.127);
#90658=CYLINDRICAL_SURFACE('',#102541,0.127000005438588);
#90659=CYLINDRICAL_SURFACE('',#102543,0.127000001278904);
#90660=CYLINDRICAL_SURFACE('',#102546,0.127);
#90661=CYLINDRICAL_SURFACE('',#102552,0.126999993613602);
#90662=CYLINDRICAL_SURFACE('',#102554,0.127000005455578);
#90663=CYLINDRICAL_SURFACE('',#102560,0.127);
#90664=CYLINDRICAL_SURFACE('',#102563,0.126999998752696);
#90665=CYLINDRICAL_SURFACE('',#102565,0.126999993594751);
#90666=CYLINDRICAL_SURFACE('',#102569,0.127);
#90667=CYLINDRICAL_SURFACE('',#102571,0.127);
#90668=CYLINDRICAL_SURFACE('',#102574,0.127000000302741);
#90669=CYLINDRICAL_SURFACE('',#102575,0.126999999706774);
#90670=CYLINDRICAL_SURFACE('',#102579,0.127);
#90671=CYLINDRICAL_SURFACE('',#102581,0.127);
#90672=CYLINDRICAL_SURFACE('',#102585,0.127000005439607);
#90673=CYLINDRICAL_SURFACE('',#102587,0.127000001278421);
#90674=CYLINDRICAL_SURFACE('',#102590,0.127);
#90675=CYLINDRICAL_SURFACE('',#102596,0.126999993617745);
#90676=CYLINDRICAL_SURFACE('',#102598,0.127000005455381);
#90677=CYLINDRICAL_SURFACE('',#102604,0.127);
#90678=CYLINDRICAL_SURFACE('',#102607,0.126999998754997);
#90679=CYLINDRICAL_SURFACE('',#102609,0.126999993595255);
#90680=CYLINDRICAL_SURFACE('',#102613,0.127);
#90681=CYLINDRICAL_SURFACE('',#102615,0.127);
#90682=CYLINDRICAL_SURFACE('',#102618,0.127000000301444);
#90683=CYLINDRICAL_SURFACE('',#102619,0.126999999706383);
#90684=CYLINDRICAL_SURFACE('',#102623,0.127);
#90685=CYLINDRICAL_SURFACE('',#102625,0.127);
#90686=CYLINDRICAL_SURFACE('',#102629,0.127000005439654);
#90687=CYLINDRICAL_SURFACE('',#102631,0.12700000127798);
#90688=CYLINDRICAL_SURFACE('',#102634,0.127);
#90689=CYLINDRICAL_SURFACE('',#102640,0.126999993615447);
#90690=CYLINDRICAL_SURFACE('',#102642,0.127000005453466);
#90691=CYLINDRICAL_SURFACE('',#102648,0.127);
#90692=CYLINDRICAL_SURFACE('',#102651,0.126999998751995);
#90693=CYLINDRICAL_SURFACE('',#102653,0.12699999359383);
#90694=CYLINDRICAL_SURFACE('',#102657,0.127);
#90695=CYLINDRICAL_SURFACE('',#102659,0.127);
#90696=CYLINDRICAL_SURFACE('',#102662,0.127000000301414);
#90697=CYLINDRICAL_SURFACE('',#102663,0.12699999970812);
#90698=CYLINDRICAL_SURFACE('',#102667,0.127);
#90699=CYLINDRICAL_SURFACE('',#102669,0.127);
#90700=CYLINDRICAL_SURFACE('',#102673,0.127000005437224);
#90701=CYLINDRICAL_SURFACE('',#102675,0.127000001279242);
#90702=CYLINDRICAL_SURFACE('',#102678,0.127);
#90703=CYLINDRICAL_SURFACE('',#102684,0.126999993612789);
#90704=CYLINDRICAL_SURFACE('',#102686,0.127000005453465);
#90705=CYLINDRICAL_SURFACE('',#102692,0.127);
#90706=CYLINDRICAL_SURFACE('',#102695,0.126999998752582);
#90707=CYLINDRICAL_SURFACE('',#102697,0.126999993593896);
#90708=CYLINDRICAL_SURFACE('',#102701,0.127);
#90709=CYLINDRICAL_SURFACE('',#102703,0.127);
#90710=CYLINDRICAL_SURFACE('',#102706,0.127000000300403);
#90711=CYLINDRICAL_SURFACE('',#102707,0.126999999707339);
#90712=CYLINDRICAL_SURFACE('',#102711,0.127);
#90713=CYLINDRICAL_SURFACE('',#102713,0.127);
#90714=CYLINDRICAL_SURFACE('',#102717,0.12700000543759);
#90715=CYLINDRICAL_SURFACE('',#102719,0.127000001278668);
#90716=CYLINDRICAL_SURFACE('',#102722,0.127);
#90717=CYLINDRICAL_SURFACE('',#102728,0.126999993616971);
#90718=CYLINDRICAL_SURFACE('',#102730,0.127000005453324);
#90719=CYLINDRICAL_SURFACE('',#102736,0.127);
#90720=CYLINDRICAL_SURFACE('',#102739,0.126999998753525);
#90721=CYLINDRICAL_SURFACE('',#102741,0.12699999359536);
#90722=CYLINDRICAL_SURFACE('',#102745,0.127);
#90723=CYLINDRICAL_SURFACE('',#102747,0.127);
#90724=CYLINDRICAL_SURFACE('',#102750,0.127000000300871);
#90725=CYLINDRICAL_SURFACE('',#102751,0.126999999706726);
#90726=CYLINDRICAL_SURFACE('',#102755,0.127);
#90727=CYLINDRICAL_SURFACE('',#102757,0.127);
#90728=CYLINDRICAL_SURFACE('',#102761,0.127000005436566);
#90729=CYLINDRICAL_SURFACE('',#102763,0.127000001279669);
#90730=CYLINDRICAL_SURFACE('',#102766,0.127);
#90731=CYLINDRICAL_SURFACE('',#102772,0.126999993612996);
#90732=CYLINDRICAL_SURFACE('',#102774,0.127000005451943);
#90733=CYLINDRICAL_SURFACE('',#102780,0.127);
#90734=CYLINDRICAL_SURFACE('',#102783,0.126999998753668);
#90735=CYLINDRICAL_SURFACE('',#102785,0.126999993597716);
#90736=CYLINDRICAL_SURFACE('',#102789,0.127);
#90737=CYLINDRICAL_SURFACE('',#102791,0.127);
#90738=CYLINDRICAL_SURFACE('',#102794,0.12700000030196);
#90739=CYLINDRICAL_SURFACE('',#102795,0.126999999706616);
#90740=CYLINDRICAL_SURFACE('',#102799,0.127);
#90741=CYLINDRICAL_SURFACE('',#102801,0.127);
#90742=CYLINDRICAL_SURFACE('',#102805,0.127000005440328);
#90743=CYLINDRICAL_SURFACE('',#102807,0.127000001279997);
#90744=CYLINDRICAL_SURFACE('',#102810,0.127);
#90745=CYLINDRICAL_SURFACE('',#102816,0.126999993614862);
#90746=CYLINDRICAL_SURFACE('',#102818,0.127000005453936);
#90747=CYLINDRICAL_SURFACE('',#102824,0.126999999999999);
#90748=CYLINDRICAL_SURFACE('',#102827,0.126999998752473);
#90749=CYLINDRICAL_SURFACE('',#102829,0.126999993593647);
#90750=CYLINDRICAL_SURFACE('',#102833,0.126999999999999);
#90751=CYLINDRICAL_SURFACE('',#102835,0.126999999999999);
#90752=CYLINDRICAL_SURFACE('',#102838,0.127000000302768);
#90753=CYLINDRICAL_SURFACE('',#102839,0.126999999706514);
#90754=CYLINDRICAL_SURFACE('',#102843,0.127);
#90755=CYLINDRICAL_SURFACE('',#102845,0.127);
#90756=CYLINDRICAL_SURFACE('',#102849,0.127000005434962);
#90757=CYLINDRICAL_SURFACE('',#102851,0.127000001278088);
#90758=CYLINDRICAL_SURFACE('',#102854,0.127);
#90759=CYLINDRICAL_SURFACE('',#102860,0.126999993617541);
#90760=CYLINDRICAL_SURFACE('',#102862,0.127000005452558);
#90761=CYLINDRICAL_SURFACE('',#102868,0.127000000000001);
#90762=CYLINDRICAL_SURFACE('',#102871,0.12699999875113);
#90763=CYLINDRICAL_SURFACE('',#102873,0.126999993594463);
#90764=CYLINDRICAL_SURFACE('',#102877,0.127000000000001);
#90765=CYLINDRICAL_SURFACE('',#102879,0.127000000000001);
#90766=CYLINDRICAL_SURFACE('',#102882,0.127000000300141);
#90767=CYLINDRICAL_SURFACE('',#102883,0.12699999970714);
#90768=CYLINDRICAL_SURFACE('',#102887,0.127);
#90769=CYLINDRICAL_SURFACE('',#102889,0.127);
#90770=CYLINDRICAL_SURFACE('',#102893,0.127000005439957);
#90771=CYLINDRICAL_SURFACE('',#102895,0.12700000127911);
#90772=CYLINDRICAL_SURFACE('',#102898,0.127);
#90773=CYLINDRICAL_SURFACE('',#102904,0.126999993615602);
#90774=CYLINDRICAL_SURFACE('',#102906,0.127000005454291);
#90775=CYLINDRICAL_SURFACE('',#102912,0.127);
#90776=CYLINDRICAL_SURFACE('',#102915,0.126999998753839);
#90777=CYLINDRICAL_SURFACE('',#102917,0.126999993595304);
#90778=CYLINDRICAL_SURFACE('',#102921,0.127);
#90779=CYLINDRICAL_SURFACE('',#102923,0.127);
#90780=CYLINDRICAL_SURFACE('',#102926,0.127000000301699);
#90781=CYLINDRICAL_SURFACE('',#102927,0.126999999705295);
#90782=CYLINDRICAL_SURFACE('',#102931,0.127);
#90783=CYLINDRICAL_SURFACE('',#102933,0.127);
#90784=CYLINDRICAL_SURFACE('',#102937,0.127000005439621);
#90785=CYLINDRICAL_SURFACE('',#102939,0.127000001279142);
#90786=CYLINDRICAL_SURFACE('',#102942,0.127);
#90787=CYLINDRICAL_SURFACE('',#102948,0.126999993614056);
#90788=CYLINDRICAL_SURFACE('',#102950,0.127000005452498);
#90789=CYLINDRICAL_SURFACE('',#102956,0.127000000000001);
#90790=CYLINDRICAL_SURFACE('',#102959,0.126999998753414);
#90791=CYLINDRICAL_SURFACE('',#102961,0.1269999935946);
#90792=CYLINDRICAL_SURFACE('',#102965,0.127000000000001);
#90793=CYLINDRICAL_SURFACE('',#102967,0.127000000000001);
#90794=CYLINDRICAL_SURFACE('',#102970,0.127000000300451);
#90795=CYLINDRICAL_SURFACE('',#102971,0.126999999707799);
#90796=CYLINDRICAL_SURFACE('',#102975,0.127);
#90797=CYLINDRICAL_SURFACE('',#102977,0.127);
#90798=CYLINDRICAL_SURFACE('',#102981,0.127000005436198);
#90799=CYLINDRICAL_SURFACE('',#102983,0.127000001278508);
#90800=CYLINDRICAL_SURFACE('',#102986,0.127);
#90801=CYLINDRICAL_SURFACE('',#102992,0.126999993613461);
#90802=CYLINDRICAL_SURFACE('',#102994,0.127000005454311);
#90803=CYLINDRICAL_SURFACE('',#103000,0.127);
#90804=CYLINDRICAL_SURFACE('',#103003,0.126999998752435);
#90805=CYLINDRICAL_SURFACE('',#103005,0.126999993594948);
#90806=CYLINDRICAL_SURFACE('',#103009,0.127);
#90807=CYLINDRICAL_SURFACE('',#103011,0.127);
#90808=CYLINDRICAL_SURFACE('',#103014,0.127000000300104);
#90809=CYLINDRICAL_SURFACE('',#103015,0.1269999997076);
#90810=CYLINDRICAL_SURFACE('',#103019,0.127);
#90811=CYLINDRICAL_SURFACE('',#103021,0.127);
#90812=CYLINDRICAL_SURFACE('',#103025,0.127000005437536);
#90813=CYLINDRICAL_SURFACE('',#103027,0.127000001280254);
#90814=CYLINDRICAL_SURFACE('',#103030,0.127);
#90815=CYLINDRICAL_SURFACE('',#103036,0.126999993616732);
#90816=CYLINDRICAL_SURFACE('',#103038,0.127000005453867);
#90817=CYLINDRICAL_SURFACE('',#103044,0.127);
#90818=CYLINDRICAL_SURFACE('',#103047,0.12699999875391);
#90819=CYLINDRICAL_SURFACE('',#103049,0.126999993592352);
#90820=CYLINDRICAL_SURFACE('',#103053,0.127);
#90821=CYLINDRICAL_SURFACE('',#103055,0.127);
#90822=CYLINDRICAL_SURFACE('',#103058,0.127000000301673);
#90823=CYLINDRICAL_SURFACE('',#103059,0.12699999970761);
#90824=CYLINDRICAL_SURFACE('',#103063,0.127);
#90825=CYLINDRICAL_SURFACE('',#103065,0.127);
#90826=CYLINDRICAL_SURFACE('',#103069,0.127000005437743);
#90827=CYLINDRICAL_SURFACE('',#103071,0.127000001277194);
#90828=CYLINDRICAL_SURFACE('',#103074,0.127);
#90829=CYLINDRICAL_SURFACE('',#103080,0.126999993615799);
#90830=CYLINDRICAL_SURFACE('',#103082,0.127000005454222);
#90831=CYLINDRICAL_SURFACE('',#103088,0.127000000000001);
#90832=CYLINDRICAL_SURFACE('',#103091,0.126999998753413);
#90833=CYLINDRICAL_SURFACE('',#103093,0.126999993594634);
#90834=CYLINDRICAL_SURFACE('',#103097,0.127000000000001);
#90835=CYLINDRICAL_SURFACE('',#103099,0.127000000000001);
#90836=CYLINDRICAL_SURFACE('',#103102,0.127000000300308);
#90837=CYLINDRICAL_SURFACE('',#103103,0.126999999707545);
#90838=CYLINDRICAL_SURFACE('',#103107,0.127);
#90839=CYLINDRICAL_SURFACE('',#103109,0.127);
#90840=CYLINDRICAL_SURFACE('',#103113,0.127000005434043);
#90841=CYLINDRICAL_SURFACE('',#103115,0.127000001279328);
#90842=CYLINDRICAL_SURFACE('',#103118,0.127);
#90843=CYLINDRICAL_SURFACE('',#103124,0.126999993613876);
#90844=CYLINDRICAL_SURFACE('',#103126,0.127000005452976);
#90845=CYLINDRICAL_SURFACE('',#103132,0.127);
#90846=CYLINDRICAL_SURFACE('',#103135,0.126999998753321);
#90847=CYLINDRICAL_SURFACE('',#103137,0.126999993597018);
#90848=CYLINDRICAL_SURFACE('',#103141,0.127);
#90849=CYLINDRICAL_SURFACE('',#103143,0.127);
#90850=CYLINDRICAL_SURFACE('',#103146,0.127000000301608);
#90851=CYLINDRICAL_SURFACE('',#103147,0.126999999705367);
#90852=CYLINDRICAL_SURFACE('',#103151,0.127);
#90853=CYLINDRICAL_SURFACE('',#103153,0.127);
#90854=CYLINDRICAL_SURFACE('',#103157,0.127000005439731);
#90855=CYLINDRICAL_SURFACE('',#103159,0.127000001277541);
#90856=CYLINDRICAL_SURFACE('',#103162,0.127);
#90857=CYLINDRICAL_SURFACE('',#103168,0.126999993617131);
#90858=CYLINDRICAL_SURFACE('',#103170,0.127000005454814);
#90859=CYLINDRICAL_SURFACE('',#103176,0.127000000000001);
#90860=CYLINDRICAL_SURFACE('',#103179,0.126999998753577);
#90861=CYLINDRICAL_SURFACE('',#103181,0.126999993598197);
#90862=CYLINDRICAL_SURFACE('',#103185,0.127000000000001);
#90863=CYLINDRICAL_SURFACE('',#103187,0.127000000000001);
#90864=CYLINDRICAL_SURFACE('',#103190,0.127000000301002);
#90865=CYLINDRICAL_SURFACE('',#103191,0.12699999970699);
#90866=CYLINDRICAL_SURFACE('',#103195,0.127);
#90867=CYLINDRICAL_SURFACE('',#103197,0.127);
#90868=CYLINDRICAL_SURFACE('',#103201,0.127000005438292);
#90869=CYLINDRICAL_SURFACE('',#103203,0.127000001278948);
#90870=CYLINDRICAL_SURFACE('',#103206,0.127);
#90871=CYLINDRICAL_SURFACE('',#103212,0.126999993613223);
#90872=CYLINDRICAL_SURFACE('',#103214,0.127000005454579);
#90873=CYLINDRICAL_SURFACE('',#103220,0.127000000000002);
#90874=CYLINDRICAL_SURFACE('',#103223,0.126999998753176);
#90875=CYLINDRICAL_SURFACE('',#103225,0.126999993594714);
#90876=CYLINDRICAL_SURFACE('',#103229,0.127000000000002);
#90877=CYLINDRICAL_SURFACE('',#103231,0.127000000000002);
#90878=CYLINDRICAL_SURFACE('',#103234,0.127000000302915);
#90879=CYLINDRICAL_SURFACE('',#103235,0.126999999706383);
#90880=CYLINDRICAL_SURFACE('',#103239,0.127);
#90881=CYLINDRICAL_SURFACE('',#103241,0.127);
#90882=CYLINDRICAL_SURFACE('',#103245,0.127000005440828);
#90883=CYLINDRICAL_SURFACE('',#103247,0.12700000127864);
#90884=CYLINDRICAL_SURFACE('',#103250,0.127);
#90885=CYLINDRICAL_SURFACE('',#103256,0.126999993616967);
#90886=CYLINDRICAL_SURFACE('',#103258,0.127000005453503);
#90887=CYLINDRICAL_SURFACE('',#103264,0.126999999999999);
#90888=CYLINDRICAL_SURFACE('',#103267,0.126999998754026);
#90889=CYLINDRICAL_SURFACE('',#103269,0.126999993593209);
#90890=CYLINDRICAL_SURFACE('',#103273,0.126999999999999);
#90891=CYLINDRICAL_SURFACE('',#103275,0.126999999999999);
#90892=CYLINDRICAL_SURFACE('',#103278,0.127000000300874);
#90893=CYLINDRICAL_SURFACE('',#103279,0.126999999706456);
#90894=CYLINDRICAL_SURFACE('',#103283,0.127);
#90895=CYLINDRICAL_SURFACE('',#103285,0.127);
#90896=CYLINDRICAL_SURFACE('',#103289,0.127000005438321);
#90897=CYLINDRICAL_SURFACE('',#103291,0.127000001279013);
#90898=CYLINDRICAL_SURFACE('',#103294,0.127);
#90899=CYLINDRICAL_SURFACE('',#103300,0.126999993615933);
#90900=CYLINDRICAL_SURFACE('',#103302,0.127000005453603);
#90901=CYLINDRICAL_SURFACE('',#103308,0.126999999999999);
#90902=CYLINDRICAL_SURFACE('',#103311,0.126999998752138);
#90903=CYLINDRICAL_SURFACE('',#103313,0.126999993597807);
#90904=CYLINDRICAL_SURFACE('',#103317,0.126999999999999);
#90905=CYLINDRICAL_SURFACE('',#103319,0.126999999999999);
#90906=CYLINDRICAL_SURFACE('',#103322,0.127000000301534);
#90907=CYLINDRICAL_SURFACE('',#103323,0.126999999705897);
#90908=CYLINDRICAL_SURFACE('',#103327,0.127000000000002);
#90909=CYLINDRICAL_SURFACE('',#103329,0.127000000000002);
#90910=CYLINDRICAL_SURFACE('',#103333,0.127000005437536);
#90911=CYLINDRICAL_SURFACE('',#103335,0.127000001278742);
#90912=CYLINDRICAL_SURFACE('',#103337,0.127000000000002);
#90913=CYLINDRICAL_SURFACE('',#103341,0.126999993615157);
#90914=CYLINDRICAL_SURFACE('',#103343,0.127000005454198);
#90915=CYLINDRICAL_SURFACE('',#103346,0.127000000000002);
#90916=CYLINDRICAL_SURFACE('',#103349,0.126999998753399);
#90917=CYLINDRICAL_SURFACE('',#103351,0.126999993594869);
#90918=CYLINDRICAL_SURFACE('',#103355,0.127000000000002);
#90919=CYLINDRICAL_SURFACE('',#103357,0.127000000000002);
#90920=CYLINDRICAL_SURFACE('',#103360,0.12700000030155);
#90921=CYLINDRICAL_SURFACE('',#103361,0.126999999707605);
#90922=CYLINDRICAL_SURFACE('',#103365,0.127);
#90923=CYLINDRICAL_SURFACE('',#103367,0.127);
#90924=CYLINDRICAL_SURFACE('',#103371,0.127000005437624);
#90925=CYLINDRICAL_SURFACE('',#103373,0.127000001279377);
#90926=CYLINDRICAL_SURFACE('',#103376,0.127);
#90927=CYLINDRICAL_SURFACE('',#103382,0.12699999361462);
#90928=CYLINDRICAL_SURFACE('',#103384,0.127000005452932);
#90929=CYLINDRICAL_SURFACE('',#103390,0.127);
#90930=CYLINDRICAL_SURFACE('',#103393,0.12699999875397);
#90931=CYLINDRICAL_SURFACE('',#103395,0.1269999935932);
#90932=CYLINDRICAL_SURFACE('',#103399,0.127);
#90933=CYLINDRICAL_SURFACE('',#103401,0.127);
#90934=CYLINDRICAL_SURFACE('',#103404,0.127000000302331);
#90935=CYLINDRICAL_SURFACE('',#103405,0.126999999708275);
#90936=CYLINDRICAL_SURFACE('',#103409,0.127);
#90937=CYLINDRICAL_SURFACE('',#103411,0.127);
#90938=CYLINDRICAL_SURFACE('',#103415,0.127000005437317);
#90939=CYLINDRICAL_SURFACE('',#103417,0.127000001278536);
#90940=CYLINDRICAL_SURFACE('',#103420,0.127);
#90941=CYLINDRICAL_SURFACE('',#103426,0.12699999361381);
#90942=CYLINDRICAL_SURFACE('',#103428,0.127000005454359);
#90943=CYLINDRICAL_SURFACE('',#103434,0.126999999999999);
#90944=CYLINDRICAL_SURFACE('',#103437,0.126999998753825);
#90945=CYLINDRICAL_SURFACE('',#103439,0.126999993596437);
#90946=CYLINDRICAL_SURFACE('',#103443,0.126999999999999);
#90947=CYLINDRICAL_SURFACE('',#103445,0.126999999999999);
#90948=CYLINDRICAL_SURFACE('',#103448,0.12700000030131);
#90949=CYLINDRICAL_SURFACE('',#103449,0.126999999705017);
#90950=CYLINDRICAL_SURFACE('',#103453,0.127);
#90951=CYLINDRICAL_SURFACE('',#103455,0.127);
#90952=CYLINDRICAL_SURFACE('',#103459,0.127000005437735);
#90953=CYLINDRICAL_SURFACE('',#103461,0.127000001278806);
#90954=CYLINDRICAL_SURFACE('',#103464,0.127);
#90955=CYLINDRICAL_SURFACE('',#103470,0.126999993614013);
#90956=CYLINDRICAL_SURFACE('',#103472,0.127000005453686);
#90957=CYLINDRICAL_SURFACE('',#103478,0.127000000000002);
#90958=CYLINDRICAL_SURFACE('',#103481,0.126999998752789);
#90959=CYLINDRICAL_SURFACE('',#103483,0.126999993596079);
#90960=CYLINDRICAL_SURFACE('',#103487,0.127000000000002);
#90961=CYLINDRICAL_SURFACE('',#103489,0.127000000000002);
#90962=CYLINDRICAL_SURFACE('',#103492,0.127000000301439);
#90963=CYLINDRICAL_SURFACE('',#103493,0.126999999704935);
#90964=CYLINDRICAL_SURFACE('',#103497,0.127);
#90965=CYLINDRICAL_SURFACE('',#103499,0.127);
#90966=CYLINDRICAL_SURFACE('',#103503,0.127000005439358);
#90967=CYLINDRICAL_SURFACE('',#103505,0.127000001277789);
#90968=CYLINDRICAL_SURFACE('',#103508,0.127);
#90969=CYLINDRICAL_SURFACE('',#103514,0.126999993617532);
#90970=CYLINDRICAL_SURFACE('',#103516,0.127000005455948);
#90971=CYLINDRICAL_SURFACE('',#103522,0.127000000000001);
#90972=CYLINDRICAL_SURFACE('',#103525,0.126999998752883);
#90973=CYLINDRICAL_SURFACE('',#103527,0.126999993593983);
#90974=CYLINDRICAL_SURFACE('',#103531,0.127000000000001);
#90975=CYLINDRICAL_SURFACE('',#103533,0.127000000000001);
#90976=CYLINDRICAL_SURFACE('',#103536,0.127000000304323);
#90977=CYLINDRICAL_SURFACE('',#103537,0.12699999970756);
#90978=CYLINDRICAL_SURFACE('',#103541,0.127);
#90979=CYLINDRICAL_SURFACE('',#103543,0.127);
#90980=CYLINDRICAL_SURFACE('',#103547,0.127000005440239);
#90981=CYLINDRICAL_SURFACE('',#103549,0.127000001279599);
#90982=CYLINDRICAL_SURFACE('',#103552,0.127);
#90983=CYLINDRICAL_SURFACE('',#103558,0.126999993612611);
#90984=CYLINDRICAL_SURFACE('',#103560,0.127000005457026);
#90985=CYLINDRICAL_SURFACE('',#103566,0.127);
#90986=CYLINDRICAL_SURFACE('',#103569,0.12699999875316);
#90987=CYLINDRICAL_SURFACE('',#103571,0.126999993596404);
#90988=CYLINDRICAL_SURFACE('',#103575,0.127);
#90989=CYLINDRICAL_SURFACE('',#103577,0.127);
#90990=CYLINDRICAL_SURFACE('',#103580,0.127000000301405);
#90991=CYLINDRICAL_SURFACE('',#103581,0.126999999707666);
#90992=CYLINDRICAL_SURFACE('',#103585,0.127);
#90993=CYLINDRICAL_SURFACE('',#103587,0.127);
#90994=CYLINDRICAL_SURFACE('',#103591,0.127000005438194);
#90995=CYLINDRICAL_SURFACE('',#103593,0.127000001279677);
#90996=CYLINDRICAL_SURFACE('',#103596,0.127);
#90997=CYLINDRICAL_SURFACE('',#103602,0.12699999361647);
#90998=CYLINDRICAL_SURFACE('',#103604,0.127000005453912);
#90999=CYLINDRICAL_SURFACE('',#103610,0.127000000000001);
#91000=CYLINDRICAL_SURFACE('',#103613,0.126999998753327);
#91001=CYLINDRICAL_SURFACE('',#103615,0.12699999359527);
#91002=CYLINDRICAL_SURFACE('',#103619,0.127000000000001);
#91003=CYLINDRICAL_SURFACE('',#103621,0.127000000000001);
#91004=CYLINDRICAL_SURFACE('',#103624,0.127000000299871);
#91005=CYLINDRICAL_SURFACE('',#103625,0.126999999705577);
#91006=CYLINDRICAL_SURFACE('',#103629,0.127);
#91007=CYLINDRICAL_SURFACE('',#103631,0.127);
#91008=CYLINDRICAL_SURFACE('',#103635,0.127000005435759);
#91009=CYLINDRICAL_SURFACE('',#103637,0.12700000127797);
#91010=CYLINDRICAL_SURFACE('',#103640,0.127);
#91011=CYLINDRICAL_SURFACE('',#103646,0.126999993612283);
#91012=CYLINDRICAL_SURFACE('',#103648,0.127000005450208);
#91013=CYLINDRICAL_SURFACE('',#103654,0.126999999999998);
#91014=CYLINDRICAL_SURFACE('',#103657,0.126999998752389);
#91015=CYLINDRICAL_SURFACE('',#103659,0.126999993595374);
#91016=CYLINDRICAL_SURFACE('',#103663,0.126999999999998);
#91017=CYLINDRICAL_SURFACE('',#103665,0.126999999999998);
#91018=CYLINDRICAL_SURFACE('',#103668,0.127000000300949);
#91019=CYLINDRICAL_SURFACE('',#103669,0.126999999707429);
#91020=CYLINDRICAL_SURFACE('',#103673,0.127);
#91021=CYLINDRICAL_SURFACE('',#103675,0.127);
#91022=CYLINDRICAL_SURFACE('',#103679,0.127000005435469);
#91023=CYLINDRICAL_SURFACE('',#103681,0.127000001280724);
#91024=CYLINDRICAL_SURFACE('',#103684,0.127);
#91025=CYLINDRICAL_SURFACE('',#103690,0.126999993616767);
#91026=CYLINDRICAL_SURFACE('',#103692,0.127000005452434);
#91027=CYLINDRICAL_SURFACE('',#103698,0.127);
#91028=CYLINDRICAL_SURFACE('',#103701,0.12699999875229);
#91029=CYLINDRICAL_SURFACE('',#103703,0.126999993596947);
#91030=CYLINDRICAL_SURFACE('',#103707,0.127);
#91031=CYLINDRICAL_SURFACE('',#103709,0.127);
#91032=CYLINDRICAL_SURFACE('',#103712,0.127000000301637);
#91033=CYLINDRICAL_SURFACE('',#103713,0.126999999707563);
#91034=CYLINDRICAL_SURFACE('',#103717,0.127);
#91035=CYLINDRICAL_SURFACE('',#103719,0.127);
#91036=CYLINDRICAL_SURFACE('',#103723,0.12700000543493);
#91037=CYLINDRICAL_SURFACE('',#103725,0.12700000127735);
#91038=CYLINDRICAL_SURFACE('',#103728,0.127);
#91039=CYLINDRICAL_SURFACE('',#103734,0.126999993615612);
#91040=CYLINDRICAL_SURFACE('',#103736,0.127000005453414);
#91041=CYLINDRICAL_SURFACE('',#103742,0.126999999999999);
#91042=CYLINDRICAL_SURFACE('',#103745,0.126999998752984);
#91043=CYLINDRICAL_SURFACE('',#103747,0.126999993593435);
#91044=CYLINDRICAL_SURFACE('',#103751,0.126999999999999);
#91045=CYLINDRICAL_SURFACE('',#103753,0.126999999999999);
#91046=CYLINDRICAL_SURFACE('',#103756,0.127000000301768);
#91047=CYLINDRICAL_SURFACE('',#103757,0.126999999706787);
#91048=CYLINDRICAL_SURFACE('',#103761,0.127);
#91049=CYLINDRICAL_SURFACE('',#103763,0.127);
#91050=CYLINDRICAL_SURFACE('',#103767,0.127000005433587);
#91051=CYLINDRICAL_SURFACE('',#103769,0.127000001278825);
#91052=CYLINDRICAL_SURFACE('',#103772,0.127);
#91053=CYLINDRICAL_SURFACE('',#103778,0.126999993613855);
#91054=CYLINDRICAL_SURFACE('',#103780,0.127000005455278);
#91055=CYLINDRICAL_SURFACE('',#103786,0.126999999999999);
#91056=CYLINDRICAL_SURFACE('',#103789,0.126999998754249);
#91057=CYLINDRICAL_SURFACE('',#103791,0.12699999359443);
#91058=CYLINDRICAL_SURFACE('',#103795,0.126999999999999);
#91059=CYLINDRICAL_SURFACE('',#103797,0.126999999999999);
#91060=CYLINDRICAL_SURFACE('',#103800,0.127000000301345);
#91061=CYLINDRICAL_SURFACE('',#103801,0.126999999707803);
#91062=CYLINDRICAL_SURFACE('',#103805,0.127);
#91063=CYLINDRICAL_SURFACE('',#103807,0.127);
#91064=CYLINDRICAL_SURFACE('',#103811,0.12700000543712);
#91065=CYLINDRICAL_SURFACE('',#103813,0.127000001279907);
#91066=CYLINDRICAL_SURFACE('',#103816,0.127);
#91067=CYLINDRICAL_SURFACE('',#103822,0.126999993614048);
#91068=CYLINDRICAL_SURFACE('',#103824,0.127000005454575);
#91069=CYLINDRICAL_SURFACE('',#103830,0.127);
#91070=CYLINDRICAL_SURFACE('',#103833,0.126999998752347);
#91071=CYLINDRICAL_SURFACE('',#103835,0.126999993597714);
#91072=CYLINDRICAL_SURFACE('',#103839,0.127);
#91073=CYLINDRICAL_SURFACE('',#103841,0.127);
#91074=CYLINDRICAL_SURFACE('',#103844,0.127000000301343);
#91075=CYLINDRICAL_SURFACE('',#103845,0.126999999707272);
#91076=CYLINDRICAL_SURFACE('',#103849,0.127);
#91077=CYLINDRICAL_SURFACE('',#103851,0.127);
#91078=CYLINDRICAL_SURFACE('',#103855,0.127000005433796);
#91079=CYLINDRICAL_SURFACE('',#103857,0.127000001278195);
#91080=CYLINDRICAL_SURFACE('',#103860,0.127);
#91081=CYLINDRICAL_SURFACE('',#103866,0.126999993613666);
#91082=CYLINDRICAL_SURFACE('',#103868,0.127000005453606);
#91083=CYLINDRICAL_SURFACE('',#103874,0.127);
#91084=CYLINDRICAL_SURFACE('',#103877,0.126999998755233);
#91085=CYLINDRICAL_SURFACE('',#103879,0.126999993596122);
#91086=CYLINDRICAL_SURFACE('',#103883,0.127);
#91087=CYLINDRICAL_SURFACE('',#103885,0.127);
#91088=CYLINDRICAL_SURFACE('',#103888,0.127000000301413);
#91089=CYLINDRICAL_SURFACE('',#103889,0.126999999707218);
#91090=CYLINDRICAL_SURFACE('',#103893,0.127);
#91091=CYLINDRICAL_SURFACE('',#103895,0.127);
#91092=CYLINDRICAL_SURFACE('',#103899,0.127000005439452);
#91093=CYLINDRICAL_SURFACE('',#103901,0.12700000127914);
#91094=CYLINDRICAL_SURFACE('',#103904,0.127);
#91095=CYLINDRICAL_SURFACE('',#103910,0.126999993615814);
#91096=CYLINDRICAL_SURFACE('',#103912,0.127000005453094);
#91097=CYLINDRICAL_SURFACE('',#103918,0.127);
#91098=CYLINDRICAL_SURFACE('',#103921,0.126999998753958);
#91099=CYLINDRICAL_SURFACE('',#103923,0.12699999359588);
#91100=CYLINDRICAL_SURFACE('',#103927,0.127);
#91101=CYLINDRICAL_SURFACE('',#103929,0.127);
#91102=CYLINDRICAL_SURFACE('',#103932,0.127000000300461);
#91103=CYLINDRICAL_SURFACE('',#103933,0.126999999706217);
#91104=CYLINDRICAL_SURFACE('',#103937,0.127);
#91105=CYLINDRICAL_SURFACE('',#103939,0.127);
#91106=CYLINDRICAL_SURFACE('',#103943,0.127000005437066);
#91107=CYLINDRICAL_SURFACE('',#103945,0.127000001279617);
#91108=CYLINDRICAL_SURFACE('',#103948,0.127);
#91109=CYLINDRICAL_SURFACE('',#103954,0.126999993615203);
#91110=CYLINDRICAL_SURFACE('',#103956,0.127000005454548);
#91111=CYLINDRICAL_SURFACE('',#103962,0.127);
#91112=CYLINDRICAL_SURFACE('',#103965,0.126999998753434);
#91113=CYLINDRICAL_SURFACE('',#103967,0.126999993595871);
#91114=CYLINDRICAL_SURFACE('',#103971,0.127);
#91115=CYLINDRICAL_SURFACE('',#103973,0.127);
#91116=CYLINDRICAL_SURFACE('',#103976,0.127000000301136);
#91117=CYLINDRICAL_SURFACE('',#103977,0.126999999708071);
#91118=CYLINDRICAL_SURFACE('',#103981,0.127);
#91119=CYLINDRICAL_SURFACE('',#103983,0.127);
#91120=CYLINDRICAL_SURFACE('',#103987,0.1270000054394);
#91121=CYLINDRICAL_SURFACE('',#103989,0.127000001278787);
#91122=CYLINDRICAL_SURFACE('',#103991,0.127);
#91123=CYLINDRICAL_SURFACE('',#103995,0.126999993612156);
#91124=CYLINDRICAL_SURFACE('',#103997,0.12700000545294);
#91125=CYLINDRICAL_SURFACE('',#104000,0.127);
#91126=CYLINDRICAL_SURFACE('',#104003,0.126999998752275);
#91127=CYLINDRICAL_SURFACE('',#104005,0.126999993594249);
#91128=CYLINDRICAL_SURFACE('',#104009,0.127);
#91129=CYLINDRICAL_SURFACE('',#104011,0.127);
#91130=CYLINDRICAL_SURFACE('',#104014,0.127000000300402);
#91131=CYLINDRICAL_SURFACE('',#104015,0.126999999707371);
#91132=CYLINDRICAL_SURFACE('',#104019,0.127);
#91133=CYLINDRICAL_SURFACE('',#104021,0.127);
#91134=CYLINDRICAL_SURFACE('',#104025,0.127000005437447);
#91135=CYLINDRICAL_SURFACE('',#104027,0.127000001277987);
#91136=CYLINDRICAL_SURFACE('',#104030,0.127);
#91137=CYLINDRICAL_SURFACE('',#104036,0.12699999361552);
#91138=CYLINDRICAL_SURFACE('',#104038,0.127000005453145);
#91139=CYLINDRICAL_SURFACE('',#104044,0.127);
#91140=CYLINDRICAL_SURFACE('',#104047,0.12699999875448);
#91141=CYLINDRICAL_SURFACE('',#104049,0.126999993595573);
#91142=CYLINDRICAL_SURFACE('',#104053,0.127);
#91143=CYLINDRICAL_SURFACE('',#104055,0.127);
#91144=CYLINDRICAL_SURFACE('',#104058,0.127000000300409);
#91145=CYLINDRICAL_SURFACE('',#104059,0.126999999706503);
#91146=CYLINDRICAL_SURFACE('',#104063,0.127);
#91147=CYLINDRICAL_SURFACE('',#104065,0.127);
#91148=CYLINDRICAL_SURFACE('',#104069,0.127000005438401);
#91149=CYLINDRICAL_SURFACE('',#104071,0.127000001278597);
#91150=CYLINDRICAL_SURFACE('',#104074,0.127);
#91151=CYLINDRICAL_SURFACE('',#104080,0.126999993616107);
#91152=CYLINDRICAL_SURFACE('',#104082,0.127000005453882);
#91153=CYLINDRICAL_SURFACE('',#104088,0.127);
#91154=CYLINDRICAL_SURFACE('',#104091,0.126999998753241);
#91155=CYLINDRICAL_SURFACE('',#104093,0.126999993597234);
#91156=CYLINDRICAL_SURFACE('',#104097,0.127);
#91157=CYLINDRICAL_SURFACE('',#104099,0.127);
#91158=CYLINDRICAL_SURFACE('',#104102,0.127000000301718);
#91159=CYLINDRICAL_SURFACE('',#104103,0.12699999970547);
#91160=CYLINDRICAL_SURFACE('',#104107,0.127);
#91161=CYLINDRICAL_SURFACE('',#104109,0.127);
#91162=CYLINDRICAL_SURFACE('',#104113,0.127000005436057);
#91163=CYLINDRICAL_SURFACE('',#104115,0.127000001278805);
#91164=CYLINDRICAL_SURFACE('',#104118,0.127);
#91165=CYLINDRICAL_SURFACE('',#104124,0.126999993612556);
#91166=CYLINDRICAL_SURFACE('',#104126,0.127000005453779);
#91167=CYLINDRICAL_SURFACE('',#104132,0.127);
#91168=CYLINDRICAL_SURFACE('',#104135,0.126999998751993);
#91169=CYLINDRICAL_SURFACE('',#104137,0.126999993594818);
#91170=CYLINDRICAL_SURFACE('',#104141,0.127);
#91171=CYLINDRICAL_SURFACE('',#104143,0.127);
#91172=CYLINDRICAL_SURFACE('',#104146,0.127000000301938);
#91173=CYLINDRICAL_SURFACE('',#104147,0.126999999706208);
#91174=CYLINDRICAL_SURFACE('',#104151,0.127);
#91175=CYLINDRICAL_SURFACE('',#104153,0.127);
#91176=CYLINDRICAL_SURFACE('',#104157,0.127000005437245);
#91177=CYLINDRICAL_SURFACE('',#104159,0.127000001279644);
#91178=CYLINDRICAL_SURFACE('',#104162,0.127);
#91179=CYLINDRICAL_SURFACE('',#104168,0.126999993611974);
#91180=CYLINDRICAL_SURFACE('',#104170,0.127000005449949);
#91181=CYLINDRICAL_SURFACE('',#104176,0.126999999999999);
#91182=CYLINDRICAL_SURFACE('',#104179,0.126999998751559);
#91183=CYLINDRICAL_SURFACE('',#104181,0.126999993594054);
#91184=CYLINDRICAL_SURFACE('',#104185,0.126999999999999);
#91185=CYLINDRICAL_SURFACE('',#104187,0.126999999999999);
#91186=CYLINDRICAL_SURFACE('',#104190,0.127000000300251);
#91187=CYLINDRICAL_SURFACE('',#104191,0.126999999705737);
#91188=CYLINDRICAL_SURFACE('',#104195,0.127);
#91189=CYLINDRICAL_SURFACE('',#104197,0.127);
#91190=CYLINDRICAL_SURFACE('',#104201,0.127000005438409);
#91191=CYLINDRICAL_SURFACE('',#104203,0.127000001278734);
#91192=CYLINDRICAL_SURFACE('',#104206,0.127);
#91193=CYLINDRICAL_SURFACE('',#104212,0.126999993613275);
#91194=CYLINDRICAL_SURFACE('',#104214,0.127000005453712);
#91195=CYLINDRICAL_SURFACE('',#104220,0.127);
#91196=CYLINDRICAL_SURFACE('',#104223,0.126999998753237);
#91197=CYLINDRICAL_SURFACE('',#104225,0.126999993593396);
#91198=CYLINDRICAL_SURFACE('',#104229,0.127);
#91199=CYLINDRICAL_SURFACE('',#104231,0.127);
#91200=CYLINDRICAL_SURFACE('',#104234,0.127000000301442);
#91201=CYLINDRICAL_SURFACE('',#104235,0.126999999706943);
#91202=CYLINDRICAL_SURFACE('',#104239,0.127);
#91203=CYLINDRICAL_SURFACE('',#104241,0.127);
#91204=CYLINDRICAL_SURFACE('',#104245,0.127000005438704);
#91205=CYLINDRICAL_SURFACE('',#104247,0.1270000012792);
#91206=CYLINDRICAL_SURFACE('',#104250,0.127);
#91207=CYLINDRICAL_SURFACE('',#104256,0.126999993618011);
#91208=CYLINDRICAL_SURFACE('',#104258,0.12700000545145);
#91209=CYLINDRICAL_SURFACE('',#104264,0.127000000000001);
#91210=CYLINDRICAL_SURFACE('',#104267,0.126999998753892);
#91211=CYLINDRICAL_SURFACE('',#104269,0.126999993593854);
#91212=CYLINDRICAL_SURFACE('',#104273,0.127000000000001);
#91213=CYLINDRICAL_SURFACE('',#104275,0.127000000000001);
#91214=CYLINDRICAL_SURFACE('',#104278,0.127000000300314);
#91215=CYLINDRICAL_SURFACE('',#104279,0.126999999707915);
#91216=CYLINDRICAL_SURFACE('',#104283,0.127);
#91217=CYLINDRICAL_SURFACE('',#104285,0.127);
#91218=CYLINDRICAL_SURFACE('',#104289,0.127000005436347);
#91219=CYLINDRICAL_SURFACE('',#104291,0.127000001279015);
#91220=CYLINDRICAL_SURFACE('',#104294,0.127);
#91221=CYLINDRICAL_SURFACE('',#104300,0.126999993613876);
#91222=CYLINDRICAL_SURFACE('',#104302,0.127000005455893);
#91223=CYLINDRICAL_SURFACE('',#104308,0.127);
#91224=CYLINDRICAL_SURFACE('',#104311,0.126999998752179);
#91225=CYLINDRICAL_SURFACE('',#104313,0.126999993595854);
#91226=CYLINDRICAL_SURFACE('',#104317,0.127);
#91227=CYLINDRICAL_SURFACE('',#104319,0.127);
#91228=CYLINDRICAL_SURFACE('',#104322,0.127000000300653);
#91229=CYLINDRICAL_SURFACE('',#104323,0.126999999706938);
#91230=CYLINDRICAL_SURFACE('',#104327,0.127);
#91231=CYLINDRICAL_SURFACE('',#104329,0.127);
#91232=CYLINDRICAL_SURFACE('',#104333,0.127000005436586);
#91233=CYLINDRICAL_SURFACE('',#104335,0.127000001280382);
#91234=CYLINDRICAL_SURFACE('',#104338,0.127);
#91235=CYLINDRICAL_SURFACE('',#104344,0.126999993617505);
#91236=CYLINDRICAL_SURFACE('',#104346,0.127000005453856);
#91237=CYLINDRICAL_SURFACE('',#104352,0.126999999999998);
#91238=CYLINDRICAL_SURFACE('',#104355,0.126999998753061);
#91239=CYLINDRICAL_SURFACE('',#104357,0.126999993592484);
#91240=CYLINDRICAL_SURFACE('',#104361,0.127);
#91241=CYLINDRICAL_SURFACE('',#104363,0.127);
#91242=CYLINDRICAL_SURFACE('',#104366,0.127000000301914);
#91243=CYLINDRICAL_SURFACE('',#104367,0.126999999708164);
#91244=CYLINDRICAL_SURFACE('',#104371,0.127);
#91245=CYLINDRICAL_SURFACE('',#104373,0.127);
#91246=CYLINDRICAL_SURFACE('',#104377,0.127000005436732);
#91247=CYLINDRICAL_SURFACE('',#104379,0.127000001278542);
#91248=CYLINDRICAL_SURFACE('',#104382,0.127);
#91249=CYLINDRICAL_SURFACE('',#104388,0.126999993613755);
#91250=CYLINDRICAL_SURFACE('',#104390,0.1270000054525);
#91251=CYLINDRICAL_SURFACE('',#104396,0.127000000000001);
#91252=CYLINDRICAL_SURFACE('',#104399,0.126999998753982);
#91253=CYLINDRICAL_SURFACE('',#104401,0.12699999359441);
#91254=CYLINDRICAL_SURFACE('',#104405,0.127000000000001);
#91255=CYLINDRICAL_SURFACE('',#104407,0.127000000000001);
#91256=CYLINDRICAL_SURFACE('',#104410,0.127000000300815);
#91257=CYLINDRICAL_SURFACE('',#104411,0.126999999707749);
#91258=CYLINDRICAL_SURFACE('',#104415,0.127);
#91259=CYLINDRICAL_SURFACE('',#104417,0.127);
#91260=CYLINDRICAL_SURFACE('',#104421,0.127000005437114);
#91261=CYLINDRICAL_SURFACE('',#104423,0.127000001278914);
#91262=CYLINDRICAL_SURFACE('',#104426,0.127);
#91263=CYLINDRICAL_SURFACE('',#104432,0.126999993615937);
#91264=CYLINDRICAL_SURFACE('',#104434,0.127000005456152);
#91265=CYLINDRICAL_SURFACE('',#104440,0.127000000000003);
#91266=CYLINDRICAL_SURFACE('',#104443,0.126999998752603);
#91267=CYLINDRICAL_SURFACE('',#104445,0.126999993596602);
#91268=CYLINDRICAL_SURFACE('',#104449,0.127000000000003);
#91269=CYLINDRICAL_SURFACE('',#104451,0.127000000000003);
#91270=CYLINDRICAL_SURFACE('',#104454,0.127000000301358);
#91271=CYLINDRICAL_SURFACE('',#104455,0.126999999706635);
#91272=CYLINDRICAL_SURFACE('',#104459,0.127);
#91273=CYLINDRICAL_SURFACE('',#104461,0.127);
#91274=CYLINDRICAL_SURFACE('',#104465,0.127000005440303);
#91275=CYLINDRICAL_SURFACE('',#104467,0.127000001277462);
#91276=CYLINDRICAL_SURFACE('',#104470,0.127);
#91277=CYLINDRICAL_SURFACE('',#104476,0.126999993614758);
#91278=CYLINDRICAL_SURFACE('',#104478,0.127000005453311);
#91279=CYLINDRICAL_SURFACE('',#104484,0.127000000000001);
#91280=CYLINDRICAL_SURFACE('',#104487,0.126999998753895);
#91281=CYLINDRICAL_SURFACE('',#104489,0.126999993594221);
#91282=CYLINDRICAL_SURFACE('',#104493,0.127000000000001);
#91283=CYLINDRICAL_SURFACE('',#104495,0.127000000000001);
#91284=CYLINDRICAL_SURFACE('',#104498,0.127000000302199);
#91285=CYLINDRICAL_SURFACE('',#104499,0.12699999970607);
#91286=CYLINDRICAL_SURFACE('',#104503,0.127);
#91287=CYLINDRICAL_SURFACE('',#104505,0.127);
#91288=CYLINDRICAL_SURFACE('',#104509,0.12700000543857);
#91289=CYLINDRICAL_SURFACE('',#104511,0.127000001278887);
#91290=CYLINDRICAL_SURFACE('',#104514,0.127);
#91291=CYLINDRICAL_SURFACE('',#104520,0.126999993614607);
#91292=CYLINDRICAL_SURFACE('',#104522,0.127000005454939);
#91293=CYLINDRICAL_SURFACE('',#104528,0.127);
#91294=CYLINDRICAL_SURFACE('',#104531,0.126999998753384);
#91295=CYLINDRICAL_SURFACE('',#104533,0.12699999359301);
#91296=CYLINDRICAL_SURFACE('',#104537,0.127);
#91297=CYLINDRICAL_SURFACE('',#104539,0.127);
#91298=CYLINDRICAL_SURFACE('',#104542,0.12700000030178);
#91299=CYLINDRICAL_SURFACE('',#104543,0.126999999706677);
#91300=CYLINDRICAL_SURFACE('',#104547,0.127);
#91301=CYLINDRICAL_SURFACE('',#104549,0.127);
#91302=CYLINDRICAL_SURFACE('',#104553,0.127000005438697);
#91303=CYLINDRICAL_SURFACE('',#104555,0.127000001277866);
#91304=CYLINDRICAL_SURFACE('',#104558,0.127);
#91305=CYLINDRICAL_SURFACE('',#104564,0.126999993613173);
#91306=CYLINDRICAL_SURFACE('',#104566,0.127000005452212);
#91307=CYLINDRICAL_SURFACE('',#104572,0.127000000000001);
#91308=CYLINDRICAL_SURFACE('',#104575,0.126999998752685);
#91309=CYLINDRICAL_SURFACE('',#104577,0.126999993595208);
#91310=CYLINDRICAL_SURFACE('',#104581,0.127000000000001);
#91311=CYLINDRICAL_SURFACE('',#104583,0.127000000000001);
#91312=CYLINDRICAL_SURFACE('',#104586,0.127000000300787);
#91313=CYLINDRICAL_SURFACE('',#104587,0.126999999705652);
#91314=CYLINDRICAL_SURFACE('',#104591,0.127);
#91315=CYLINDRICAL_SURFACE('',#104593,0.127);
#91316=CYLINDRICAL_SURFACE('',#104597,0.127000005437709);
#91317=CYLINDRICAL_SURFACE('',#104599,0.127000001279523);
#91318=CYLINDRICAL_SURFACE('',#104602,0.127);
#91319=CYLINDRICAL_SURFACE('',#104608,0.126999993615976);
#91320=CYLINDRICAL_SURFACE('',#104610,0.127000005453785);
#91321=CYLINDRICAL_SURFACE('',#104616,0.126999999999999);
#91322=CYLINDRICAL_SURFACE('',#104619,0.126999998753079);
#91323=CYLINDRICAL_SURFACE('',#104621,0.126999993596377);
#91324=CYLINDRICAL_SURFACE('',#104625,0.126999999999999);
#91325=CYLINDRICAL_SURFACE('',#104627,0.126999999999999);
#91326=CYLINDRICAL_SURFACE('',#104630,0.12700000030257);
#91327=CYLINDRICAL_SURFACE('',#104670,65.);
#91328=CYLINDRICAL_SURFACE('',#104916,56.875);
#91329=CYLINDRICAL_SURFACE('',#106674,0.17526);
#91330=CYLINDRICAL_SURFACE('',#106675,0.17526);
#91331=CYLINDRICAL_SURFACE('',#106676,0.126999999705986);
#91332=CYLINDRICAL_SURFACE('',#106680,0.127);
#91333=CYLINDRICAL_SURFACE('',#106682,0.127);
#91334=CYLINDRICAL_SURFACE('',#106686,0.127000005436524);
#91335=CYLINDRICAL_SURFACE('',#106688,0.127000001280155);
#91336=CYLINDRICAL_SURFACE('',#106691,0.127);
#91337=CYLINDRICAL_SURFACE('',#106697,0.126999993615336);
#91338=CYLINDRICAL_SURFACE('',#106699,0.127000005452344);
#91339=CYLINDRICAL_SURFACE('',#106705,0.127);
#91340=CYLINDRICAL_SURFACE('',#106708,0.126999998752966);
#91341=CYLINDRICAL_SURFACE('',#106710,0.126999993594016);
#91342=CYLINDRICAL_SURFACE('',#106714,0.127);
#91343=CYLINDRICAL_SURFACE('',#106716,0.127);
#91344=CYLINDRICAL_SURFACE('',#106719,0.127000000300436);
#91345=CYLINDRICAL_SURFACE('',#107483,0.175259999999999);
#91346=CYLINDRICAL_SURFACE('',#107484,0.17526);
#91347=CYLINDRICAL_SURFACE('',#107485,0.175259999999999);
#91348=CYLINDRICAL_SURFACE('',#107486,0.17526);
#91349=CYLINDRICAL_SURFACE('',#107487,0.175259999999999);
#91350=CYLINDRICAL_SURFACE('',#107488,0.17526);
#91351=CYLINDRICAL_SURFACE('',#107489,0.17526);
#91352=CYLINDRICAL_SURFACE('',#107490,0.17526);
#91353=CYLINDRICAL_SURFACE('',#107491,0.175259999999998);
#91354=CYLINDRICAL_SURFACE('',#107492,0.17526);
#91355=CYLINDRICAL_SURFACE('',#107493,0.17526);
#91356=CYLINDRICAL_SURFACE('',#107494,0.17526);
#91357=CYLINDRICAL_SURFACE('',#107495,0.175260000000001);
#91358=CYLINDRICAL_SURFACE('',#107496,0.17526);
#91359=CYLINDRICAL_SURFACE('',#107497,0.175260000000001);
#91360=CYLINDRICAL_SURFACE('',#107498,0.17526);
#91361=CYLINDRICAL_SURFACE('',#107499,0.17526);
#91362=CYLINDRICAL_SURFACE('',#107500,0.17526);
#91363=CYLINDRICAL_SURFACE('',#107501,0.175260000000001);
#91364=CYLINDRICAL_SURFACE('',#107502,0.17526);
#91365=CYLINDRICAL_SURFACE('',#107503,0.17526);
#91366=CYLINDRICAL_SURFACE('',#107504,0.17526);
#91367=CYLINDRICAL_SURFACE('',#107505,0.175259999999999);
#91368=CYLINDRICAL_SURFACE('',#107506,0.17526);
#91369=CYLINDRICAL_SURFACE('',#107507,0.175259999999999);
#91370=CYLINDRICAL_SURFACE('',#107508,0.17526);
#91371=CYLINDRICAL_SURFACE('',#107509,0.175259999999999);
#91372=CYLINDRICAL_SURFACE('',#107510,0.17526);
#91373=CYLINDRICAL_SURFACE('',#107511,0.17526);
#91374=CYLINDRICAL_SURFACE('',#107512,0.17526);
#91375=CYLINDRICAL_SURFACE('',#107513,0.175259999999999);
#91376=CYLINDRICAL_SURFACE('',#107514,0.17526);
#91377=CYLINDRICAL_SURFACE('',#107515,0.17526);
#91378=CYLINDRICAL_SURFACE('',#107516,0.17526);
#91379=CYLINDRICAL_SURFACE('',#107517,0.175259999999999);
#91380=CYLINDRICAL_SURFACE('',#107518,0.17526);
#91381=CYLINDRICAL_SURFACE('',#107519,0.17526);
#91382=CYLINDRICAL_SURFACE('',#107520,0.17526);
#91383=CYLINDRICAL_SURFACE('',#107521,0.175259999999998);
#91384=CYLINDRICAL_SURFACE('',#107522,0.17526);
#91385=CYLINDRICAL_SURFACE('',#107523,0.17526);
#91386=CYLINDRICAL_SURFACE('',#107524,0.17526);
#91387=CYLINDRICAL_SURFACE('',#107525,0.175260000000001);
#91388=CYLINDRICAL_SURFACE('',#107526,0.17526);
#91389=CYLINDRICAL_SURFACE('',#107527,0.175260000000001);
#91390=CYLINDRICAL_SURFACE('',#107528,0.17526);
#91391=CYLINDRICAL_SURFACE('',#107529,0.17526);
#91392=CYLINDRICAL_SURFACE('',#107530,0.17526);
#91393=CYLINDRICAL_SURFACE('',#107531,0.175260000000001);
#91394=CYLINDRICAL_SURFACE('',#107532,0.17526);
#91395=CYLINDRICAL_SURFACE('',#107533,0.175260000000003);
#91396=CYLINDRICAL_SURFACE('',#107534,0.17526);
#91397=CYLINDRICAL_SURFACE('',#107535,0.175259999999999);
#91398=CYLINDRICAL_SURFACE('',#107536,0.17526);
#91399=CYLINDRICAL_SURFACE('',#107537,0.175259999999999);
#91400=CYLINDRICAL_SURFACE('',#107538,0.17526);
#91401=CYLINDRICAL_SURFACE('',#107539,0.17526);
#91402=CYLINDRICAL_SURFACE('',#107540,0.17526);
#91403=CYLINDRICAL_SURFACE('',#107541,0.17526);
#91404=CYLINDRICAL_SURFACE('',#107542,0.17526);
#91405=CYLINDRICAL_SURFACE('',#107543,0.17526);
#91406=CYLINDRICAL_SURFACE('',#107544,0.17526);
#91407=CYLINDRICAL_SURFACE('',#107545,0.17526);
#91408=CYLINDRICAL_SURFACE('',#107546,0.17526);
#91409=CYLINDRICAL_SURFACE('',#107547,0.175259999999999);
#91410=CYLINDRICAL_SURFACE('',#107548,0.17526);
#91411=CYLINDRICAL_SURFACE('',#107549,0.17526);
#91412=CYLINDRICAL_SURFACE('',#107550,0.17526);
#91413=CYLINDRICAL_SURFACE('',#107551,0.175259999999998);
#91414=CYLINDRICAL_SURFACE('',#107552,0.17526);
#91415=CYLINDRICAL_SURFACE('',#107553,0.17526);
#91416=CYLINDRICAL_SURFACE('',#107554,0.17526);
#91417=CYLINDRICAL_SURFACE('',#107555,0.175259999999996);
#91418=CYLINDRICAL_SURFACE('',#107556,0.17526);
#91419=CYLINDRICAL_SURFACE('',#107557,0.175260000000001);
#91420=CYLINDRICAL_SURFACE('',#107558,0.17526);
#91421=CYLINDRICAL_SURFACE('',#107559,0.175259999999995);
#91422=CYLINDRICAL_SURFACE('',#107560,0.17526);
#91423=CYLINDRICAL_SURFACE('',#107561,0.175260000000001);
#91424=CYLINDRICAL_SURFACE('',#107562,0.17526);
#91425=CYLINDRICAL_SURFACE('',#107563,0.17526);
#91426=CYLINDRICAL_SURFACE('',#107564,0.17526);
#91427=CYLINDRICAL_SURFACE('',#107565,0.175259999999999);
#91428=CYLINDRICAL_SURFACE('',#107566,0.17526);
#91429=CYLINDRICAL_SURFACE('',#107567,0.175259999999999);
#91430=CYLINDRICAL_SURFACE('',#107568,0.17526);
#91431=CYLINDRICAL_SURFACE('',#107569,0.17526);
#91432=CYLINDRICAL_SURFACE('',#107570,0.17526);
#91433=CYLINDRICAL_SURFACE('',#107571,0.17526);
#91434=CYLINDRICAL_SURFACE('',#107572,0.17526);
#91435=CYLINDRICAL_SURFACE('',#107573,0.17526);
#91436=CYLINDRICAL_SURFACE('',#107574,0.17526);
#91437=CYLINDRICAL_SURFACE('',#107575,0.17526);
#91438=CYLINDRICAL_SURFACE('',#107576,0.17526);
#91439=CYLINDRICAL_SURFACE('',#107577,0.175259999999999);
#91440=CYLINDRICAL_SURFACE('',#107578,0.17526);
#91441=CYLINDRICAL_SURFACE('',#107579,0.17526);
#91442=CYLINDRICAL_SURFACE('',#107580,0.17526);
#91443=CYLINDRICAL_SURFACE('',#107581,0.175260000000001);
#91444=CYLINDRICAL_SURFACE('',#107582,0.17526);
#91445=CYLINDRICAL_SURFACE('',#107583,0.17526);
#91446=CYLINDRICAL_SURFACE('',#107584,0.17526);
#91447=CYLINDRICAL_SURFACE('',#107585,0.175259999999996);
#91448=CYLINDRICAL_SURFACE('',#107586,0.17526);
#91449=CYLINDRICAL_SURFACE('',#107587,0.175260000000001);
#91450=CYLINDRICAL_SURFACE('',#107588,0.17526);
#91451=CYLINDRICAL_SURFACE('',#107589,0.175260000000001);
#91452=CYLINDRICAL_SURFACE('',#107590,0.17526);
#91453=CYLINDRICAL_SURFACE('',#107591,0.175260000000001);
#91454=CYLINDRICAL_SURFACE('',#107592,0.17526);
#91455=CYLINDRICAL_SURFACE('',#107593,0.17526);
#91456=CYLINDRICAL_SURFACE('',#107594,0.17526);
#91457=CYLINDRICAL_SURFACE('',#107595,0.175259999999999);
#91458=CYLINDRICAL_SURFACE('',#107596,0.17526);
#91459=CYLINDRICAL_SURFACE('',#107597,0.175259999999999);
#91460=CYLINDRICAL_SURFACE('',#107598,0.17526);
#91461=CYLINDRICAL_SURFACE('',#107599,0.17526);
#91462=CYLINDRICAL_SURFACE('',#107600,0.17526);
#91463=CYLINDRICAL_SURFACE('',#107601,0.126999999705659);
#91464=CYLINDRICAL_SURFACE('',#107605,0.127);
#91465=CYLINDRICAL_SURFACE('',#107607,0.127);
#91466=CYLINDRICAL_SURFACE('',#107611,0.127000005438804);
#91467=CYLINDRICAL_SURFACE('',#107613,0.127000001278595);
#91468=CYLINDRICAL_SURFACE('',#107616,0.127);
#91469=CYLINDRICAL_SURFACE('',#107622,0.126999993613258);
#91470=CYLINDRICAL_SURFACE('',#107624,0.127000005456531);
#91471=CYLINDRICAL_SURFACE('',#107630,0.126999999999999);
#91472=CYLINDRICAL_SURFACE('',#107633,0.126999998754334);
#91473=CYLINDRICAL_SURFACE('',#107635,0.126999993594558);
#91474=CYLINDRICAL_SURFACE('',#107639,0.126999999999999);
#91475=CYLINDRICAL_SURFACE('',#107641,0.126999999999999);
#91476=CYLINDRICAL_SURFACE('',#107644,0.127000000302017);
#91477=CYLINDRICAL_SURFACE('',#107645,0.126999999706877);
#91478=CYLINDRICAL_SURFACE('',#107649,0.127);
#91479=CYLINDRICAL_SURFACE('',#107651,0.127);
#91480=CYLINDRICAL_SURFACE('',#107655,0.127000005438286);
#91481=CYLINDRICAL_SURFACE('',#107657,0.127000001280016);
#91482=CYLINDRICAL_SURFACE('',#107660,0.127);
#91483=CYLINDRICAL_SURFACE('',#107666,0.126999993612901);
#91484=CYLINDRICAL_SURFACE('',#107668,0.127000005452847);
#91485=CYLINDRICAL_SURFACE('',#107674,0.126999999999999);
#91486=CYLINDRICAL_SURFACE('',#107677,0.12699999875172);
#91487=CYLINDRICAL_SURFACE('',#107679,0.126999993595217);
#91488=CYLINDRICAL_SURFACE('',#107683,0.126999999999999);
#91489=CYLINDRICAL_SURFACE('',#107685,0.126999999999999);
#91490=CYLINDRICAL_SURFACE('',#107688,0.127000000302727);
#91491=CYLINDRICAL_SURFACE('',#107689,0.126999999707438);
#91492=CYLINDRICAL_SURFACE('',#107693,0.127);
#91493=CYLINDRICAL_SURFACE('',#107695,0.127);
#91494=CYLINDRICAL_SURFACE('',#107699,0.127000005439645);
#91495=CYLINDRICAL_SURFACE('',#107701,0.127000001279045);
#91496=CYLINDRICAL_SURFACE('',#107704,0.127);
#91497=CYLINDRICAL_SURFACE('',#107710,0.126999993613143);
#91498=CYLINDRICAL_SURFACE('',#107712,0.127000005454004);
#91499=CYLINDRICAL_SURFACE('',#107718,0.127000000000002);
#91500=CYLINDRICAL_SURFACE('',#107721,0.126999998753197);
#91501=CYLINDRICAL_SURFACE('',#107723,0.126999993594632);
#91502=CYLINDRICAL_SURFACE('',#107727,0.127000000000002);
#91503=CYLINDRICAL_SURFACE('',#107729,0.127000000000002);
#91504=CYLINDRICAL_SURFACE('',#107732,0.127000000302894);
#91505=CYLINDRICAL_SURFACE('',#107733,0.126999999705007);
#91506=CYLINDRICAL_SURFACE('',#107737,0.127);
#91507=CYLINDRICAL_SURFACE('',#107739,0.127);
#91508=CYLINDRICAL_SURFACE('',#107743,0.127000005436761);
#91509=CYLINDRICAL_SURFACE('',#107745,0.127000001278623);
#91510=CYLINDRICAL_SURFACE('',#107748,0.127);
#91511=CYLINDRICAL_SURFACE('',#107754,0.126999993614452);
#91512=CYLINDRICAL_SURFACE('',#107756,0.127000005456074);
#91513=CYLINDRICAL_SURFACE('',#107762,0.127000000000001);
#91514=CYLINDRICAL_SURFACE('',#107765,0.126999998753102);
#91515=CYLINDRICAL_SURFACE('',#107767,0.126999993593139);
#91516=CYLINDRICAL_SURFACE('',#107771,0.127000000000001);
#91517=CYLINDRICAL_SURFACE('',#107773,0.127000000000001);
#91518=CYLINDRICAL_SURFACE('',#107776,0.127000000302033);
#91519=CYLINDRICAL_SURFACE('',#107777,0.126999999705891);
#91520=CYLINDRICAL_SURFACE('',#107781,0.127);
#91521=CYLINDRICAL_SURFACE('',#107783,0.127);
#91522=CYLINDRICAL_SURFACE('',#107787,0.127000005438578);
#91523=CYLINDRICAL_SURFACE('',#107789,0.127000001278986);
#91524=CYLINDRICAL_SURFACE('',#107792,0.127);
#91525=CYLINDRICAL_SURFACE('',#107798,0.126999993613499);
#91526=CYLINDRICAL_SURFACE('',#107800,0.127000005452666);
#91527=CYLINDRICAL_SURFACE('',#107806,0.127);
#91528=CYLINDRICAL_SURFACE('',#107809,0.1269999987535);
#91529=CYLINDRICAL_SURFACE('',#107811,0.126999993594111);
#91530=CYLINDRICAL_SURFACE('',#107815,0.127);
#91531=CYLINDRICAL_SURFACE('',#107817,0.127);
#91532=CYLINDRICAL_SURFACE('',#107820,0.127000000301114);
#91533=CYLINDRICAL_SURFACE('',#107821,0.126999999706381);
#91534=CYLINDRICAL_SURFACE('',#107825,0.127);
#91535=CYLINDRICAL_SURFACE('',#107827,0.127);
#91536=CYLINDRICAL_SURFACE('',#107831,0.127000005437376);
#91537=CYLINDRICAL_SURFACE('',#107833,0.12700000127869);
#91538=CYLINDRICAL_SURFACE('',#107836,0.127);
#91539=CYLINDRICAL_SURFACE('',#107842,0.126999993614952);
#91540=CYLINDRICAL_SURFACE('',#107844,0.127000005452941);
#91541=CYLINDRICAL_SURFACE('',#107850,0.127000000000001);
#91542=CYLINDRICAL_SURFACE('',#107853,0.126999998752931);
#91543=CYLINDRICAL_SURFACE('',#107855,0.126999993591758);
#91544=CYLINDRICAL_SURFACE('',#107859,0.127000000000001);
#91545=CYLINDRICAL_SURFACE('',#107861,0.127000000000001);
#91546=CYLINDRICAL_SURFACE('',#107864,0.127000000300221);
#91547=CYLINDRICAL_SURFACE('',#107865,0.126999999706944);
#91548=CYLINDRICAL_SURFACE('',#107869,0.127);
#91549=CYLINDRICAL_SURFACE('',#107871,0.127);
#91550=CYLINDRICAL_SURFACE('',#107875,0.127000005438498);
#91551=CYLINDRICAL_SURFACE('',#107877,0.127000001278942);
#91552=CYLINDRICAL_SURFACE('',#107880,0.127);
#91553=CYLINDRICAL_SURFACE('',#107886,0.126999993619589);
#91554=CYLINDRICAL_SURFACE('',#107888,0.12700000545362);
#91555=CYLINDRICAL_SURFACE('',#107894,0.126999999999998);
#91556=CYLINDRICAL_SURFACE('',#107897,0.12699999875288);
#91557=CYLINDRICAL_SURFACE('',#107899,0.126999993594423);
#91558=CYLINDRICAL_SURFACE('',#107903,0.126999999999998);
#91559=CYLINDRICAL_SURFACE('',#107905,0.126999999999998);
#91560=CYLINDRICAL_SURFACE('',#107908,0.127000000302494);
#91561=CYLINDRICAL_SURFACE('',#107909,0.126999999707788);
#91562=CYLINDRICAL_SURFACE('',#107913,0.127);
#91563=CYLINDRICAL_SURFACE('',#107915,0.127);
#91564=CYLINDRICAL_SURFACE('',#107919,0.127000005437275);
#91565=CYLINDRICAL_SURFACE('',#107921,0.127000001280034);
#91566=CYLINDRICAL_SURFACE('',#107924,0.127);
#91567=CYLINDRICAL_SURFACE('',#107930,0.126999993614549);
#91568=CYLINDRICAL_SURFACE('',#107932,0.127000005453645);
#91569=CYLINDRICAL_SURFACE('',#107938,0.127);
#91570=CYLINDRICAL_SURFACE('',#107941,0.126999998753375);
#91571=CYLINDRICAL_SURFACE('',#107943,0.126999993593803);
#91572=CYLINDRICAL_SURFACE('',#107947,0.127);
#91573=CYLINDRICAL_SURFACE('',#107949,0.127);
#91574=CYLINDRICAL_SURFACE('',#107952,0.127000000302309);
#91575=CYLINDRICAL_SURFACE('',#107953,0.126999999706647);
#91576=CYLINDRICAL_SURFACE('',#107957,0.127);
#91577=CYLINDRICAL_SURFACE('',#107959,0.127);
#91578=CYLINDRICAL_SURFACE('',#107963,0.127000005438832);
#91579=CYLINDRICAL_SURFACE('',#107965,0.127000001280675);
#91580=CYLINDRICAL_SURFACE('',#107968,0.127);
#91581=CYLINDRICAL_SURFACE('',#107974,0.126999993615939);
#91582=CYLINDRICAL_SURFACE('',#107976,0.12700000545297);
#91583=CYLINDRICAL_SURFACE('',#107982,0.126999999999999);
#91584=CYLINDRICAL_SURFACE('',#107985,0.126999998754127);
#91585=CYLINDRICAL_SURFACE('',#107987,0.126999993593799);
#91586=CYLINDRICAL_SURFACE('',#107991,0.126999999999999);
#91587=CYLINDRICAL_SURFACE('',#107993,0.126999999999999);
#91588=CYLINDRICAL_SURFACE('',#107996,0.12700000030121);
#91589=CYLINDRICAL_SURFACE('',#107997,0.126999999706712);
#91590=CYLINDRICAL_SURFACE('',#108001,0.127);
#91591=CYLINDRICAL_SURFACE('',#108003,0.127);
#91592=CYLINDRICAL_SURFACE('',#108007,0.127000005438327);
#91593=CYLINDRICAL_SURFACE('',#108009,0.127000001279818);
#91594=CYLINDRICAL_SURFACE('',#108012,0.127);
#91595=CYLINDRICAL_SURFACE('',#108018,0.126999993613333);
#91596=CYLINDRICAL_SURFACE('',#108020,0.127000005454714);
#91597=CYLINDRICAL_SURFACE('',#108026,0.127);
#91598=CYLINDRICAL_SURFACE('',#108029,0.126999998752385);
#91599=CYLINDRICAL_SURFACE('',#108031,0.126999993595799);
#91600=CYLINDRICAL_SURFACE('',#108035,0.127000000000001);
#91601=CYLINDRICAL_SURFACE('',#108037,0.127000000000001);
#91602=CYLINDRICAL_SURFACE('',#108040,0.12700000030205);
#91603=CYLINDRICAL_SURFACE('',#108041,0.126999999707271);
#91604=CYLINDRICAL_SURFACE('',#108045,0.127);
#91605=CYLINDRICAL_SURFACE('',#108047,0.127);
#91606=CYLINDRICAL_SURFACE('',#108051,0.127000005437262);
#91607=CYLINDRICAL_SURFACE('',#108053,0.127000001277901);
#91608=CYLINDRICAL_SURFACE('',#108056,0.127);
#91609=CYLINDRICAL_SURFACE('',#108062,0.126999993615953);
#91610=CYLINDRICAL_SURFACE('',#108064,0.127000005455153);
#91611=CYLINDRICAL_SURFACE('',#108070,0.127000000000001);
#91612=CYLINDRICAL_SURFACE('',#108073,0.126999998754757);
#91613=CYLINDRICAL_SURFACE('',#108075,0.12699999359852);
#91614=CYLINDRICAL_SURFACE('',#108079,0.127000000000001);
#91615=CYLINDRICAL_SURFACE('',#108081,0.127000000000001);
#91616=CYLINDRICAL_SURFACE('',#108084,0.127000000302116);
#91617=CYLINDRICAL_SURFACE('',#108085,0.126999999707366);
#91618=CYLINDRICAL_SURFACE('',#108089,0.127);
#91619=CYLINDRICAL_SURFACE('',#108091,0.127);
#91620=CYLINDRICAL_SURFACE('',#108095,0.127000005434585);
#91621=CYLINDRICAL_SURFACE('',#108097,0.127000001280038);
#91622=CYLINDRICAL_SURFACE('',#108100,0.127);
#91623=CYLINDRICAL_SURFACE('',#108106,0.126999993613355);
#91624=CYLINDRICAL_SURFACE('',#108108,0.127000005454191);
#91625=CYLINDRICAL_SURFACE('',#108114,0.127);
#91626=CYLINDRICAL_SURFACE('',#108117,0.126999998752333);
#91627=CYLINDRICAL_SURFACE('',#108119,0.126999993594576);
#91628=CYLINDRICAL_SURFACE('',#108123,0.127);
#91629=CYLINDRICAL_SURFACE('',#108125,0.127);
#91630=CYLINDRICAL_SURFACE('',#108128,0.127000000300596);
#91631=CYLINDRICAL_SURFACE('',#108129,0.126999999707311);
#91632=CYLINDRICAL_SURFACE('',#108133,0.127);
#91633=CYLINDRICAL_SURFACE('',#108135,0.127);
#91634=CYLINDRICAL_SURFACE('',#108139,0.127000005439773);
#91635=CYLINDRICAL_SURFACE('',#108141,0.127000001277871);
#91636=CYLINDRICAL_SURFACE('',#108144,0.127);
#91637=CYLINDRICAL_SURFACE('',#108150,0.126999993616715);
#91638=CYLINDRICAL_SURFACE('',#108152,0.127000005452816);
#91639=CYLINDRICAL_SURFACE('',#108158,0.127);
#91640=CYLINDRICAL_SURFACE('',#108161,0.126999998753913);
#91641=CYLINDRICAL_SURFACE('',#108163,0.126999993595481);
#91642=CYLINDRICAL_SURFACE('',#108167,0.127);
#91643=CYLINDRICAL_SURFACE('',#108169,0.127);
#91644=CYLINDRICAL_SURFACE('',#108172,0.127000000300196);
#91645=CYLINDRICAL_SURFACE('',#108173,0.126999999705456);
#91646=CYLINDRICAL_SURFACE('',#108177,0.127);
#91647=CYLINDRICAL_SURFACE('',#108179,0.127);
#91648=CYLINDRICAL_SURFACE('',#108183,0.127000005436537);
#91649=CYLINDRICAL_SURFACE('',#108185,0.12700000127896);
#91650=CYLINDRICAL_SURFACE('',#108188,0.127);
#91651=CYLINDRICAL_SURFACE('',#108194,0.126999993615659);
#91652=CYLINDRICAL_SURFACE('',#108196,0.127000005453786);
#91653=CYLINDRICAL_SURFACE('',#108202,0.127);
#91654=CYLINDRICAL_SURFACE('',#108205,0.12699999875271);
#91655=CYLINDRICAL_SURFACE('',#108207,0.126999993596784);
#91656=CYLINDRICAL_SURFACE('',#108211,0.127);
#91657=CYLINDRICAL_SURFACE('',#108213,0.127);
#91658=CYLINDRICAL_SURFACE('',#108216,0.127000000301125);
#91659=CYLINDRICAL_SURFACE('',#108217,0.126999999707381);
#91660=CYLINDRICAL_SURFACE('',#108221,0.127);
#91661=CYLINDRICAL_SURFACE('',#108223,0.127);
#91662=CYLINDRICAL_SURFACE('',#108227,0.127000005436994);
#91663=CYLINDRICAL_SURFACE('',#108229,0.127000001279189);
#91664=CYLINDRICAL_SURFACE('',#108232,0.127);
#91665=CYLINDRICAL_SURFACE('',#108238,0.126999993613671);
#91666=CYLINDRICAL_SURFACE('',#108240,0.127000005453692);
#91667=CYLINDRICAL_SURFACE('',#108246,0.127);
#91668=CYLINDRICAL_SURFACE('',#108249,0.126999998754202);
#91669=CYLINDRICAL_SURFACE('',#108251,0.126999993593398);
#91670=CYLINDRICAL_SURFACE('',#108255,0.127);
#91671=CYLINDRICAL_SURFACE('',#108257,0.127);
#91672=CYLINDRICAL_SURFACE('',#108260,0.127000000301612);
#91673=CYLINDRICAL_SURFACE('',#108261,0.126999999706848);
#91674=CYLINDRICAL_SURFACE('',#108265,0.127);
#91675=CYLINDRICAL_SURFACE('',#108267,0.127);
#91676=CYLINDRICAL_SURFACE('',#108271,0.127000005437153);
#91677=CYLINDRICAL_SURFACE('',#108273,0.127000001278536);
#91678=CYLINDRICAL_SURFACE('',#108276,0.127);
#91679=CYLINDRICAL_SURFACE('',#108282,0.126999993614016);
#91680=CYLINDRICAL_SURFACE('',#108284,0.127000005452352);
#91681=CYLINDRICAL_SURFACE('',#108290,0.127);
#91682=CYLINDRICAL_SURFACE('',#108293,0.126999998753935);
#91683=CYLINDRICAL_SURFACE('',#108295,0.126999993594902);
#91684=CYLINDRICAL_SURFACE('',#108299,0.127);
#91685=CYLINDRICAL_SURFACE('',#108301,0.127);
#91686=CYLINDRICAL_SURFACE('',#108304,0.127000000300736);
#91687=CYLINDRICAL_SURFACE('',#108305,0.126999999706529);
#91688=CYLINDRICAL_SURFACE('',#108309,0.127);
#91689=CYLINDRICAL_SURFACE('',#108311,0.127);
#91690=CYLINDRICAL_SURFACE('',#108315,0.127000005438594);
#91691=CYLINDRICAL_SURFACE('',#108317,0.127000001279977);
#91692=CYLINDRICAL_SURFACE('',#108320,0.127);
#91693=CYLINDRICAL_SURFACE('',#108326,0.126999993615537);
#91694=CYLINDRICAL_SURFACE('',#108328,0.127000005452522);
#91695=CYLINDRICAL_SURFACE('',#108334,0.127);
#91696=CYLINDRICAL_SURFACE('',#108337,0.126999998752468);
#91697=CYLINDRICAL_SURFACE('',#108339,0.126999993596773);
#91698=CYLINDRICAL_SURFACE('',#108343,0.127);
#91699=CYLINDRICAL_SURFACE('',#108345,0.127);
#91700=CYLINDRICAL_SURFACE('',#108348,0.127000000301443);
#91701=CYLINDRICAL_SURFACE('',#108349,0.126999999704752);
#91702=CYLINDRICAL_SURFACE('',#108353,0.127);
#91703=CYLINDRICAL_SURFACE('',#108355,0.127);
#91704=CYLINDRICAL_SURFACE('',#108359,0.127000005440182);
#91705=CYLINDRICAL_SURFACE('',#108361,0.127000001279415);
#91706=CYLINDRICAL_SURFACE('',#108364,0.127);
#91707=CYLINDRICAL_SURFACE('',#108370,0.12699999361407);
#91708=CYLINDRICAL_SURFACE('',#108372,0.127000005453498);
#91709=CYLINDRICAL_SURFACE('',#108378,0.126999999999999);
#91710=CYLINDRICAL_SURFACE('',#108381,0.126999998753558);
#91711=CYLINDRICAL_SURFACE('',#108383,0.126999993595186);
#91712=CYLINDRICAL_SURFACE('',#108387,0.126999999999999);
#91713=CYLINDRICAL_SURFACE('',#108389,0.126999999999999);
#91714=CYLINDRICAL_SURFACE('',#108392,0.127000000302269);
#91715=CYLINDRICAL_SURFACE('',#108393,0.126999999706853);
#91716=CYLINDRICAL_SURFACE('',#108397,0.127);
#91717=CYLINDRICAL_SURFACE('',#108399,0.127);
#91718=CYLINDRICAL_SURFACE('',#108403,0.127000005436064);
#91719=CYLINDRICAL_SURFACE('',#108405,0.127000001278517);
#91720=CYLINDRICAL_SURFACE('',#108408,0.127);
#91721=CYLINDRICAL_SURFACE('',#108414,0.126999993620423);
#91722=CYLINDRICAL_SURFACE('',#108416,0.127000005452903);
#91723=CYLINDRICAL_SURFACE('',#108422,0.127000000000001);
#91724=CYLINDRICAL_SURFACE('',#108425,0.126999998753051);
#91725=CYLINDRICAL_SURFACE('',#108427,0.126999993597228);
#91726=CYLINDRICAL_SURFACE('',#108431,0.127000000000001);
#91727=CYLINDRICAL_SURFACE('',#108433,0.127000000000001);
#91728=CYLINDRICAL_SURFACE('',#108436,0.127000000301954);
#91729=CYLINDRICAL_SURFACE('',#108437,0.126999999706396);
#91730=CYLINDRICAL_SURFACE('',#108441,0.127);
#91731=CYLINDRICAL_SURFACE('',#108443,0.127);
#91732=CYLINDRICAL_SURFACE('',#108447,0.127000005437226);
#91733=CYLINDRICAL_SURFACE('',#108449,0.127000001279001);
#91734=CYLINDRICAL_SURFACE('',#108452,0.127);
#91735=CYLINDRICAL_SURFACE('',#108458,0.12699999361601);
#91736=CYLINDRICAL_SURFACE('',#108460,0.127000005455446);
#91737=CYLINDRICAL_SURFACE('',#108466,0.127);
#91738=CYLINDRICAL_SURFACE('',#108469,0.126999998753164);
#91739=CYLINDRICAL_SURFACE('',#108471,0.126999993595105);
#91740=CYLINDRICAL_SURFACE('',#108475,0.127);
#91741=CYLINDRICAL_SURFACE('',#108477,0.127);
#91742=CYLINDRICAL_SURFACE('',#108480,0.12700000030132);
#91743=CYLINDRICAL_SURFACE('',#108481,0.126999999705817);
#91744=CYLINDRICAL_SURFACE('',#108485,0.127);
#91745=CYLINDRICAL_SURFACE('',#108487,0.127);
#91746=CYLINDRICAL_SURFACE('',#108491,0.127000005439081);
#91747=CYLINDRICAL_SURFACE('',#108493,0.127000001278701);
#91748=CYLINDRICAL_SURFACE('',#108496,0.127);
#91749=CYLINDRICAL_SURFACE('',#108502,0.12699999361471);
#91750=CYLINDRICAL_SURFACE('',#108504,0.127000005455995);
#91751=CYLINDRICAL_SURFACE('',#108510,0.127000000000001);
#91752=CYLINDRICAL_SURFACE('',#108513,0.126999998754023);
#91753=CYLINDRICAL_SURFACE('',#108515,0.126999993595822);
#91754=CYLINDRICAL_SURFACE('',#108519,0.127000000000001);
#91755=CYLINDRICAL_SURFACE('',#108521,0.127000000000001);
#91756=CYLINDRICAL_SURFACE('',#108524,0.127000000300876);
#91757=CYLINDRICAL_SURFACE('',#108525,0.126999999707033);
#91758=CYLINDRICAL_SURFACE('',#108529,0.127);
#91759=CYLINDRICAL_SURFACE('',#108531,0.127);
#91760=CYLINDRICAL_SURFACE('',#108535,0.127000005440277);
#91761=CYLINDRICAL_SURFACE('',#108537,0.127000001277889);
#91762=CYLINDRICAL_SURFACE('',#108540,0.127);
#91763=CYLINDRICAL_SURFACE('',#108546,0.126999993612714);
#91764=CYLINDRICAL_SURFACE('',#108548,0.127000005448686);
#91765=CYLINDRICAL_SURFACE('',#108554,0.127);
#91766=CYLINDRICAL_SURFACE('',#108557,0.126999998752826);
#91767=CYLINDRICAL_SURFACE('',#108559,0.126999993595237);
#91768=CYLINDRICAL_SURFACE('',#108563,0.127);
#91769=CYLINDRICAL_SURFACE('',#108565,0.127);
#91770=CYLINDRICAL_SURFACE('',#108568,0.127000000300549);
#91771=CYLINDRICAL_SURFACE('',#108569,0.126999999706643);
#91772=CYLINDRICAL_SURFACE('',#108573,0.127);
#91773=CYLINDRICAL_SURFACE('',#108575,0.127);
#91774=CYLINDRICAL_SURFACE('',#108579,0.127000005436435);
#91775=CYLINDRICAL_SURFACE('',#108581,0.127000001281433);
#91776=CYLINDRICAL_SURFACE('',#108584,0.127);
#91777=CYLINDRICAL_SURFACE('',#108590,0.126999993613013);
#91778=CYLINDRICAL_SURFACE('',#108592,0.127000005453951);
#91779=CYLINDRICAL_SURFACE('',#108598,0.127);
#91780=CYLINDRICAL_SURFACE('',#108601,0.126999998753876);
#91781=CYLINDRICAL_SURFACE('',#108603,0.126999993592809);
#91782=CYLINDRICAL_SURFACE('',#108607,0.127);
#91783=CYLINDRICAL_SURFACE('',#108609,0.127);
#91784=CYLINDRICAL_SURFACE('',#108612,0.127000000301689);
#91785=CYLINDRICAL_SURFACE('',#108613,0.126999999707302);
#91786=CYLINDRICAL_SURFACE('',#108617,0.127);
#91787=CYLINDRICAL_SURFACE('',#108619,0.127);
#91788=CYLINDRICAL_SURFACE('',#108623,0.127000005436606);
#91789=CYLINDRICAL_SURFACE('',#108625,0.127000001276832);
#91790=CYLINDRICAL_SURFACE('',#108628,0.127);
#91791=CYLINDRICAL_SURFACE('',#108634,0.126999993613542);
#91792=CYLINDRICAL_SURFACE('',#108636,0.127000005453435);
#91793=CYLINDRICAL_SURFACE('',#108642,0.127000000000001);
#91794=CYLINDRICAL_SURFACE('',#108645,0.126999998753528);
#91795=CYLINDRICAL_SURFACE('',#108647,0.126999993595165);
#91796=CYLINDRICAL_SURFACE('',#108651,0.127000000000001);
#91797=CYLINDRICAL_SURFACE('',#108653,0.127000000000001);
#91798=CYLINDRICAL_SURFACE('',#108656,0.127000000300756);
#91799=CYLINDRICAL_SURFACE('',#108657,0.126999999707029);
#91800=CYLINDRICAL_SURFACE('',#108661,0.127);
#91801=CYLINDRICAL_SURFACE('',#108663,0.127);
#91802=CYLINDRICAL_SURFACE('',#108667,0.127000005435516);
#91803=CYLINDRICAL_SURFACE('',#108669,0.127000001278317);
#91804=CYLINDRICAL_SURFACE('',#108672,0.127);
#91805=CYLINDRICAL_SURFACE('',#108678,0.126999993613955);
#91806=CYLINDRICAL_SURFACE('',#108680,0.127000005452699);
#91807=CYLINDRICAL_SURFACE('',#108686,0.127);
#91808=CYLINDRICAL_SURFACE('',#108689,0.126999998753515);
#91809=CYLINDRICAL_SURFACE('',#108691,0.126999993596424);
#91810=CYLINDRICAL_SURFACE('',#108695,0.127);
#91811=CYLINDRICAL_SURFACE('',#108697,0.127);
#91812=CYLINDRICAL_SURFACE('',#108700,0.127000000301871);
#91813=CYLINDRICAL_SURFACE('',#108701,0.126999999706675);
#91814=CYLINDRICAL_SURFACE('',#108705,0.127);
#91815=CYLINDRICAL_SURFACE('',#108707,0.127);
#91816=CYLINDRICAL_SURFACE('',#108711,0.127000005439049);
#91817=CYLINDRICAL_SURFACE('',#108713,0.127000001277567);
#91818=CYLINDRICAL_SURFACE('',#108716,0.127);
#91819=CYLINDRICAL_SURFACE('',#108722,0.12699999361663);
#91820=CYLINDRICAL_SURFACE('',#108724,0.127000005453719);
#91821=CYLINDRICAL_SURFACE('',#108730,0.127000000000001);
#91822=CYLINDRICAL_SURFACE('',#108733,0.126999998751427);
#91823=CYLINDRICAL_SURFACE('',#108735,0.126999993596735);
#91824=CYLINDRICAL_SURFACE('',#108739,0.127000000000001);
#91825=CYLINDRICAL_SURFACE('',#108741,0.127000000000001);
#91826=CYLINDRICAL_SURFACE('',#108744,0.127000000301557);
#91827=CYLINDRICAL_SURFACE('',#108745,0.126999999707433);
#91828=CYLINDRICAL_SURFACE('',#108749,0.127);
#91829=CYLINDRICAL_SURFACE('',#108751,0.127);
#91830=CYLINDRICAL_SURFACE('',#108755,0.127000005437756);
#91831=CYLINDRICAL_SURFACE('',#108757,0.127000001278296);
#91832=CYLINDRICAL_SURFACE('',#108760,0.127);
#91833=CYLINDRICAL_SURFACE('',#108766,0.126999993613017);
#91834=CYLINDRICAL_SURFACE('',#108768,0.127000005454635);
#91835=CYLINDRICAL_SURFACE('',#108774,0.127000000000002);
#91836=CYLINDRICAL_SURFACE('',#108777,0.126999998753502);
#91837=CYLINDRICAL_SURFACE('',#108779,0.126999993595);
#91838=CYLINDRICAL_SURFACE('',#108783,0.127000000000002);
#91839=CYLINDRICAL_SURFACE('',#108785,0.127000000000002);
#91840=CYLINDRICAL_SURFACE('',#108788,0.127000000302929);
#91841=CYLINDRICAL_SURFACE('',#108789,0.126999999706685);
#91842=CYLINDRICAL_SURFACE('',#108793,0.127);
#91843=CYLINDRICAL_SURFACE('',#108795,0.127);
#91844=CYLINDRICAL_SURFACE('',#108799,0.127000005439371);
#91845=CYLINDRICAL_SURFACE('',#108801,0.127000001278466);
#91846=CYLINDRICAL_SURFACE('',#108804,0.127);
#91847=CYLINDRICAL_SURFACE('',#108810,0.126999993615652);
#91848=CYLINDRICAL_SURFACE('',#108812,0.127000005453095);
#91849=CYLINDRICAL_SURFACE('',#108818,0.126999999999999);
#91850=CYLINDRICAL_SURFACE('',#108821,0.126999998752404);
#91851=CYLINDRICAL_SURFACE('',#108823,0.126999993593318);
#91852=CYLINDRICAL_SURFACE('',#108827,0.126999999999999);
#91853=CYLINDRICAL_SURFACE('',#108829,0.126999999999999);
#91854=CYLINDRICAL_SURFACE('',#108832,0.12700000030076);
#91855=CYLINDRICAL_SURFACE('',#108833,0.126999999706931);
#91856=CYLINDRICAL_SURFACE('',#108837,0.127);
#91857=CYLINDRICAL_SURFACE('',#108839,0.127);
#91858=CYLINDRICAL_SURFACE('',#108843,0.127000005438782);
#91859=CYLINDRICAL_SURFACE('',#108845,0.127000001278968);
#91860=CYLINDRICAL_SURFACE('',#108848,0.127);
#91861=CYLINDRICAL_SURFACE('',#108854,0.126999993616082);
#91862=CYLINDRICAL_SURFACE('',#108856,0.127000005452452);
#91863=CYLINDRICAL_SURFACE('',#108862,0.126999999999999);
#91864=CYLINDRICAL_SURFACE('',#108865,0.126999998751743);
#91865=CYLINDRICAL_SURFACE('',#108867,0.126999993596233);
#91866=CYLINDRICAL_SURFACE('',#108871,0.126999999999999);
#91867=CYLINDRICAL_SURFACE('',#108873,0.126999999999999);
#91868=CYLINDRICAL_SURFACE('',#108876,0.127000000301475);
#91869=CYLINDRICAL_SURFACE('',#108877,0.126999999707036);
#91870=CYLINDRICAL_SURFACE('',#108881,0.127);
#91871=CYLINDRICAL_SURFACE('',#108883,0.127);
#91872=CYLINDRICAL_SURFACE('',#108887,0.12700000543752);
#91873=CYLINDRICAL_SURFACE('',#108889,0.12700000127917);
#91874=CYLINDRICAL_SURFACE('',#108891,0.127);
#91875=CYLINDRICAL_SURFACE('',#108895,0.126999993614675);
#91876=CYLINDRICAL_SURFACE('',#108897,0.127000005454215);
#91877=CYLINDRICAL_SURFACE('',#108900,0.127);
#91878=CYLINDRICAL_SURFACE('',#108903,0.126999998753483);
#91879=CYLINDRICAL_SURFACE('',#108905,0.126999993594397);
#91880=CYLINDRICAL_SURFACE('',#108909,0.127);
#91881=CYLINDRICAL_SURFACE('',#108911,0.127);
#91882=CYLINDRICAL_SURFACE('',#108914,0.12700000030073);
#91883=CYLINDRICAL_SURFACE('',#108915,0.126999999707031);
#91884=CYLINDRICAL_SURFACE('',#108919,0.127);
#91885=CYLINDRICAL_SURFACE('',#108921,0.127);
#91886=CYLINDRICAL_SURFACE('',#108925,0.127000005436211);
#91887=CYLINDRICAL_SURFACE('',#108927,0.127000001279552);
#91888=CYLINDRICAL_SURFACE('',#108930,0.127);
#91889=CYLINDRICAL_SURFACE('',#108936,0.12699999361449);
#91890=CYLINDRICAL_SURFACE('',#108938,0.127000005453587);
#91891=CYLINDRICAL_SURFACE('',#108944,0.127);
#91892=CYLINDRICAL_SURFACE('',#108947,0.126999998754038);
#91893=CYLINDRICAL_SURFACE('',#108949,0.1269999935941);
#91894=CYLINDRICAL_SURFACE('',#108953,0.127);
#91895=CYLINDRICAL_SURFACE('',#108955,0.127);
#91896=CYLINDRICAL_SURFACE('',#108958,0.127000000302173);
#91897=CYLINDRICAL_SURFACE('',#108959,0.126999999706813);
#91898=CYLINDRICAL_SURFACE('',#108963,0.127);
#91899=CYLINDRICAL_SURFACE('',#108965,0.127);
#91900=CYLINDRICAL_SURFACE('',#108969,0.127000005436503);
#91901=CYLINDRICAL_SURFACE('',#108971,0.127000001279098);
#91902=CYLINDRICAL_SURFACE('',#108974,0.127);
#91903=CYLINDRICAL_SURFACE('',#108980,0.126999993612834);
#91904=CYLINDRICAL_SURFACE('',#108982,0.127000005453372);
#91905=CYLINDRICAL_SURFACE('',#108988,0.126999999999999);
#91906=CYLINDRICAL_SURFACE('',#108991,0.126999998753505);
#91907=CYLINDRICAL_SURFACE('',#108993,0.126999993596201);
#91908=CYLINDRICAL_SURFACE('',#108997,0.126999999999999);
#91909=CYLINDRICAL_SURFACE('',#108999,0.126999999999999);
#91910=CYLINDRICAL_SURFACE('',#109002,0.127000000301212);
#91911=CYLINDRICAL_SURFACE('',#109003,0.126999999705899);
#91912=CYLINDRICAL_SURFACE('',#109007,0.127);
#91913=CYLINDRICAL_SURFACE('',#109009,0.127);
#91914=CYLINDRICAL_SURFACE('',#109013,0.127000005438409);
#91915=CYLINDRICAL_SURFACE('',#109015,0.127000001279442);
#91916=CYLINDRICAL_SURFACE('',#109018,0.127);
#91917=CYLINDRICAL_SURFACE('',#109024,0.12699999361406);
#91918=CYLINDRICAL_SURFACE('',#109026,0.127000005452943);
#91919=CYLINDRICAL_SURFACE('',#109032,0.127000000000002);
#91920=CYLINDRICAL_SURFACE('',#109035,0.126999998753321);
#91921=CYLINDRICAL_SURFACE('',#109037,0.126999993595877);
#91922=CYLINDRICAL_SURFACE('',#109041,0.127000000000002);
#91923=CYLINDRICAL_SURFACE('',#109043,0.127000000000002);
#91924=CYLINDRICAL_SURFACE('',#109046,0.127000000299965);
#91925=CYLINDRICAL_SURFACE('',#109047,0.126999999705897);
#91926=CYLINDRICAL_SURFACE('',#109051,0.127);
#91927=CYLINDRICAL_SURFACE('',#109053,0.127);
#91928=CYLINDRICAL_SURFACE('',#109057,0.127000005435509);
#91929=CYLINDRICAL_SURFACE('',#109059,0.127000001277923);
#91930=CYLINDRICAL_SURFACE('',#109062,0.127);
#91931=CYLINDRICAL_SURFACE('',#109068,0.126999993617466);
#91932=CYLINDRICAL_SURFACE('',#109070,0.127000005455358);
#91933=CYLINDRICAL_SURFACE('',#109076,0.127000000000001);
#91934=CYLINDRICAL_SURFACE('',#109079,0.126999998752887);
#91935=CYLINDRICAL_SURFACE('',#109081,0.126999993594245);
#91936=CYLINDRICAL_SURFACE('',#109085,0.127000000000001);
#91937=CYLINDRICAL_SURFACE('',#109087,0.127000000000001);
#91938=CYLINDRICAL_SURFACE('',#109090,0.127000000304167);
#91939=CYLINDRICAL_SURFACE('',#109091,0.126999999706985);
#91940=CYLINDRICAL_SURFACE('',#109095,0.127);
#91941=CYLINDRICAL_SURFACE('',#109097,0.127);
#91942=CYLINDRICAL_SURFACE('',#109101,0.127000005438515);
#91943=CYLINDRICAL_SURFACE('',#109103,0.127000001279855);
#91944=CYLINDRICAL_SURFACE('',#109106,0.127);
#91945=CYLINDRICAL_SURFACE('',#109112,0.126999993613953);
#91946=CYLINDRICAL_SURFACE('',#109114,0.127000005453777);
#91947=CYLINDRICAL_SURFACE('',#109120,0.127);
#91948=CYLINDRICAL_SURFACE('',#109123,0.126999998753514);
#91949=CYLINDRICAL_SURFACE('',#109125,0.126999993595633);
#91950=CYLINDRICAL_SURFACE('',#109129,0.127);
#91951=CYLINDRICAL_SURFACE('',#109131,0.127);
#91952=CYLINDRICAL_SURFACE('',#109134,0.127000000301529);
#91953=CYLINDRICAL_SURFACE('',#109135,0.126999999707782);
#91954=CYLINDRICAL_SURFACE('',#109139,0.127);
#91955=CYLINDRICAL_SURFACE('',#109141,0.127);
#91956=CYLINDRICAL_SURFACE('',#109145,0.127000005438866);
#91957=CYLINDRICAL_SURFACE('',#109147,0.127000001278808);
#91958=CYLINDRICAL_SURFACE('',#109150,0.127);
#91959=CYLINDRICAL_SURFACE('',#109156,0.126999993614064);
#91960=CYLINDRICAL_SURFACE('',#109158,0.127000005456815);
#91961=CYLINDRICAL_SURFACE('',#109164,0.127000000000001);
#91962=CYLINDRICAL_SURFACE('',#109167,0.126999998754654);
#91963=CYLINDRICAL_SURFACE('',#109169,0.126999993594296);
#91964=CYLINDRICAL_SURFACE('',#109173,0.127000000000001);
#91965=CYLINDRICAL_SURFACE('',#109175,0.127000000000001);
#91966=CYLINDRICAL_SURFACE('',#109178,0.127000000300983);
#91967=CYLINDRICAL_SURFACE('',#109179,0.126999999705392);
#91968=CYLINDRICAL_SURFACE('',#109183,0.127);
#91969=CYLINDRICAL_SURFACE('',#109185,0.127);
#91970=CYLINDRICAL_SURFACE('',#109189,0.127000005439403);
#91971=CYLINDRICAL_SURFACE('',#109191,0.127000001278241);
#91972=CYLINDRICAL_SURFACE('',#109194,0.127);
#91973=CYLINDRICAL_SURFACE('',#109200,0.126999993613067);
#91974=CYLINDRICAL_SURFACE('',#109202,0.127000005450225);
#91975=CYLINDRICAL_SURFACE('',#109208,0.127);
#91976=CYLINDRICAL_SURFACE('',#109211,0.126999998752507);
#91977=CYLINDRICAL_SURFACE('',#109213,0.126999993595906);
#91978=CYLINDRICAL_SURFACE('',#109217,0.126999999999998);
#91979=CYLINDRICAL_SURFACE('',#109219,0.126999999999998);
#91980=CYLINDRICAL_SURFACE('',#109222,0.127000000300819);
#91981=CYLINDRICAL_SURFACE('',#109223,0.12699999970718);
#91982=CYLINDRICAL_SURFACE('',#109227,0.127);
#91983=CYLINDRICAL_SURFACE('',#109229,0.127);
#91984=CYLINDRICAL_SURFACE('',#109233,0.127000005439627);
#91985=CYLINDRICAL_SURFACE('',#109235,0.127000001280374);
#91986=CYLINDRICAL_SURFACE('',#109238,0.127);
#91987=CYLINDRICAL_SURFACE('',#109244,0.126999993617036);
#91988=CYLINDRICAL_SURFACE('',#109246,0.127000005455582);
#91989=CYLINDRICAL_SURFACE('',#109252,0.127);
#91990=CYLINDRICAL_SURFACE('',#109255,0.126999998754372);
#91991=CYLINDRICAL_SURFACE('',#109257,0.126999993594177);
#91992=CYLINDRICAL_SURFACE('',#109261,0.127);
#91993=CYLINDRICAL_SURFACE('',#109263,0.127);
#91994=CYLINDRICAL_SURFACE('',#109266,0.127000000302369);
#91995=CYLINDRICAL_SURFACE('',#109267,0.126999999707532);
#91996=CYLINDRICAL_SURFACE('',#109271,0.127);
#91997=CYLINDRICAL_SURFACE('',#109273,0.127);
#91998=CYLINDRICAL_SURFACE('',#109277,0.127000005437497);
#91999=CYLINDRICAL_SURFACE('',#109279,0.127000001277774);
#92000=CYLINDRICAL_SURFACE('',#109282,0.127);
#92001=CYLINDRICAL_SURFACE('',#109288,0.126999993612577);
#92002=CYLINDRICAL_SURFACE('',#109290,0.127000005453578);
#92003=CYLINDRICAL_SURFACE('',#109296,0.126999999999999);
#92004=CYLINDRICAL_SURFACE('',#109299,0.126999998752716);
#92005=CYLINDRICAL_SURFACE('',#109301,0.126999993596218);
#92006=CYLINDRICAL_SURFACE('',#109305,0.126999999999999);
#92007=CYLINDRICAL_SURFACE('',#109307,0.126999999999999);
#92008=CYLINDRICAL_SURFACE('',#109310,0.127000000300701);
#92009=CYLINDRICAL_SURFACE('',#109311,0.1269999997065);
#92010=CYLINDRICAL_SURFACE('',#109315,0.127);
#92011=CYLINDRICAL_SURFACE('',#109317,0.127);
#92012=CYLINDRICAL_SURFACE('',#109321,0.127000005436142);
#92013=CYLINDRICAL_SURFACE('',#109323,0.127000001277649);
#92014=CYLINDRICAL_SURFACE('',#109326,0.127);
#92015=CYLINDRICAL_SURFACE('',#109332,0.126999993613931);
#92016=CYLINDRICAL_SURFACE('',#109334,0.127000005454595);
#92017=CYLINDRICAL_SURFACE('',#109340,0.126999999999999);
#92018=CYLINDRICAL_SURFACE('',#109343,0.126999998752409);
#92019=CYLINDRICAL_SURFACE('',#109345,0.126999993591051);
#92020=CYLINDRICAL_SURFACE('',#109349,0.126999999999999);
#92021=CYLINDRICAL_SURFACE('',#109351,0.126999999999999);
#92022=CYLINDRICAL_SURFACE('',#109354,0.127000000301064);
#92023=CYLINDRICAL_SURFACE('',#109355,0.126999999706341);
#92024=CYLINDRICAL_SURFACE('',#109359,0.127);
#92025=CYLINDRICAL_SURFACE('',#109361,0.127);
#92026=CYLINDRICAL_SURFACE('',#109365,0.127000005438825);
#92027=CYLINDRICAL_SURFACE('',#109367,0.12700000127896);
#92028=CYLINDRICAL_SURFACE('',#109370,0.127);
#92029=CYLINDRICAL_SURFACE('',#109376,0.12699999361487);
#92030=CYLINDRICAL_SURFACE('',#109378,0.127000005452653);
#92031=CYLINDRICAL_SURFACE('',#109384,0.127);
#92032=CYLINDRICAL_SURFACE('',#109387,0.126999998753426);
#92033=CYLINDRICAL_SURFACE('',#109389,0.126999993597575);
#92034=CYLINDRICAL_SURFACE('',#109393,0.127);
#92035=CYLINDRICAL_SURFACE('',#109395,0.127);
#92036=CYLINDRICAL_SURFACE('',#109398,0.127000000301659);
#92037=CYLINDRICAL_SURFACE('',#109399,0.126999999707843);
#92038=CYLINDRICAL_SURFACE('',#109403,0.127);
#92039=CYLINDRICAL_SURFACE('',#109405,0.127);
#92040=CYLINDRICAL_SURFACE('',#109409,0.127000005437191);
#92041=CYLINDRICAL_SURFACE('',#109411,0.127000001278864);
#92042=CYLINDRICAL_SURFACE('',#109414,0.127);
#92043=CYLINDRICAL_SURFACE('',#109420,0.126999993613427);
#92044=CYLINDRICAL_SURFACE('',#109422,0.12700000545429);
#92045=CYLINDRICAL_SURFACE('',#109428,0.127);
#92046=CYLINDRICAL_SURFACE('',#109431,0.126999998753965);
#92047=CYLINDRICAL_SURFACE('',#109433,0.126999993595399);
#92048=CYLINDRICAL_SURFACE('',#109437,0.127);
#92049=CYLINDRICAL_SURFACE('',#109439,0.127);
#92050=CYLINDRICAL_SURFACE('',#109442,0.127000000301173);
#92051=CYLINDRICAL_SURFACE('',#109443,0.126999999708117);
#92052=CYLINDRICAL_SURFACE('',#109447,0.127);
#92053=CYLINDRICAL_SURFACE('',#109449,0.127);
#92054=CYLINDRICAL_SURFACE('',#109453,0.127000005437342);
#92055=CYLINDRICAL_SURFACE('',#109455,0.127000001278195);
#92056=CYLINDRICAL_SURFACE('',#109458,0.127);
#92057=CYLINDRICAL_SURFACE('',#109464,0.126999993615767);
#92058=CYLINDRICAL_SURFACE('',#109466,0.127000005451853);
#92059=CYLINDRICAL_SURFACE('',#109472,0.127);
#92060=CYLINDRICAL_SURFACE('',#109475,0.126999998752689);
#92061=CYLINDRICAL_SURFACE('',#109477,0.126999993594723);
#92062=CYLINDRICAL_SURFACE('',#109481,0.127);
#92063=CYLINDRICAL_SURFACE('',#109483,0.127);
#92064=CYLINDRICAL_SURFACE('',#109486,0.127000000299924);
#92065=CYLINDRICAL_SURFACE('',#109487,0.126999999704618);
#92066=CYLINDRICAL_SURFACE('',#109491,0.127);
#92067=CYLINDRICAL_SURFACE('',#109493,0.127);
#92068=CYLINDRICAL_SURFACE('',#109497,0.127000005435034);
#92069=CYLINDRICAL_SURFACE('',#109499,0.127000001280224);
#92070=CYLINDRICAL_SURFACE('',#109502,0.127);
#92071=CYLINDRICAL_SURFACE('',#109508,0.126999993615577);
#92072=CYLINDRICAL_SURFACE('',#109510,0.127000005454888);
#92073=CYLINDRICAL_SURFACE('',#109516,0.127);
#92074=CYLINDRICAL_SURFACE('',#109519,0.126999998753446);
#92075=CYLINDRICAL_SURFACE('',#109521,0.12699999359529);
#92076=CYLINDRICAL_SURFACE('',#109525,0.127);
#92077=CYLINDRICAL_SURFACE('',#109527,0.127);
#92078=CYLINDRICAL_SURFACE('',#109530,0.127000000301916);
#92079=CYLINDRICAL_SURFACE('',#109531,0.126999999705462);
#92080=CYLINDRICAL_SURFACE('',#109535,0.127);
#92081=CYLINDRICAL_SURFACE('',#109537,0.127);
#92082=CYLINDRICAL_SURFACE('',#109541,0.127000005439802);
#92083=CYLINDRICAL_SURFACE('',#109543,0.127000001278521);
#92084=CYLINDRICAL_SURFACE('',#109545,0.127);
#92085=CYLINDRICAL_SURFACE('',#109549,0.126999993615003);
#92086=CYLINDRICAL_SURFACE('',#109551,0.12700000545229);
#92087=CYLINDRICAL_SURFACE('',#109554,0.127);
#92088=CYLINDRICAL_SURFACE('',#109557,0.126999998753605);
#92089=CYLINDRICAL_SURFACE('',#109559,0.126999993595434);
#92090=CYLINDRICAL_SURFACE('',#109563,0.127);
#92091=CYLINDRICAL_SURFACE('',#109565,0.127);
#92092=CYLINDRICAL_SURFACE('',#109568,0.127000000301634);
#92093=CYLINDRICAL_SURFACE('',#109569,0.126999999706563);
#92094=CYLINDRICAL_SURFACE('',#109573,0.127);
#92095=CYLINDRICAL_SURFACE('',#109575,0.127);
#92096=CYLINDRICAL_SURFACE('',#109579,0.127000005437472);
#92097=CYLINDRICAL_SURFACE('',#109581,0.127000001278037);
#92098=CYLINDRICAL_SURFACE('',#109584,0.127);
#92099=CYLINDRICAL_SURFACE('',#109590,0.126999993614555);
#92100=CYLINDRICAL_SURFACE('',#109592,0.127000005454137);
#92101=CYLINDRICAL_SURFACE('',#109598,0.127);
#92102=CYLINDRICAL_SURFACE('',#109601,0.126999998754154);
#92103=CYLINDRICAL_SURFACE('',#109603,0.126999993593391);
#92104=CYLINDRICAL_SURFACE('',#109607,0.127);
#92105=CYLINDRICAL_SURFACE('',#109609,0.127);
#92106=CYLINDRICAL_SURFACE('',#109612,0.12700000030181);
#92107=CYLINDRICAL_SURFACE('',#109613,0.126999999708026);
#92108=CYLINDRICAL_SURFACE('',#109617,0.127);
#92109=CYLINDRICAL_SURFACE('',#109619,0.127);
#92110=CYLINDRICAL_SURFACE('',#109623,0.12700000543711);
#92111=CYLINDRICAL_SURFACE('',#109625,0.127000001279361);
#92112=CYLINDRICAL_SURFACE('',#109628,0.127);
#92113=CYLINDRICAL_SURFACE('',#109634,0.126999993615229);
#92114=CYLINDRICAL_SURFACE('',#109636,0.127000005453427);
#92115=CYLINDRICAL_SURFACE('',#109642,0.127);
#92116=CYLINDRICAL_SURFACE('',#109645,0.126999998752725);
#92117=CYLINDRICAL_SURFACE('',#109647,0.126999993597096);
#92118=CYLINDRICAL_SURFACE('',#109651,0.127);
#92119=CYLINDRICAL_SURFACE('',#109653,0.127);
#92120=CYLINDRICAL_SURFACE('',#109656,0.127000000301725);
#92121=CYLINDRICAL_SURFACE('',#109657,0.126999999706422);
#92122=CYLINDRICAL_SURFACE('',#109661,0.127);
#92123=CYLINDRICAL_SURFACE('',#109663,0.127);
#92124=CYLINDRICAL_SURFACE('',#109667,0.127000005439341);
#92125=CYLINDRICAL_SURFACE('',#109669,0.127000001278882);
#92126=CYLINDRICAL_SURFACE('',#109672,0.127);
#92127=CYLINDRICAL_SURFACE('',#109678,0.126999993613762);
#92128=CYLINDRICAL_SURFACE('',#109680,0.127000005452003);
#92129=CYLINDRICAL_SURFACE('',#109686,0.127);
#92130=CYLINDRICAL_SURFACE('',#109689,0.126999998752492);
#92131=CYLINDRICAL_SURFACE('',#109691,0.12699999359364);
#92132=CYLINDRICAL_SURFACE('',#109695,0.127);
#92133=CYLINDRICAL_SURFACE('',#109697,0.127);
#92134=CYLINDRICAL_SURFACE('',#109700,0.127000000300672);
#92135=CYLINDRICAL_SURFACE('',#109701,0.126999999705238);
#92136=CYLINDRICAL_SURFACE('',#109705,0.127);
#92137=CYLINDRICAL_SURFACE('',#109707,0.127);
#92138=CYLINDRICAL_SURFACE('',#109711,0.127000005436153);
#92139=CYLINDRICAL_SURFACE('',#109713,0.127000001278167);
#92140=CYLINDRICAL_SURFACE('',#109716,0.127);
#92141=CYLINDRICAL_SURFACE('',#109722,0.126999993615688);
#92142=CYLINDRICAL_SURFACE('',#109724,0.127000005455986);
#92143=CYLINDRICAL_SURFACE('',#109730,0.126999999999999);
#92144=CYLINDRICAL_SURFACE('',#109733,0.126999998752203);
#92145=CYLINDRICAL_SURFACE('',#109735,0.126999993593721);
#92146=CYLINDRICAL_SURFACE('',#109739,0.126999999999999);
#92147=CYLINDRICAL_SURFACE('',#109741,0.126999999999999);
#92148=CYLINDRICAL_SURFACE('',#109744,0.127000000302232);
#92149=CYLINDRICAL_SURFACE('',#109745,0.126999999704091);
#92150=CYLINDRICAL_SURFACE('',#109749,0.127);
#92151=CYLINDRICAL_SURFACE('',#109751,0.127);
#92152=CYLINDRICAL_SURFACE('',#109755,0.127000005437327);
#92153=CYLINDRICAL_SURFACE('',#109757,0.127000001279529);
#92154=CYLINDRICAL_SURFACE('',#109760,0.127);
#92155=CYLINDRICAL_SURFACE('',#109766,0.126999993615739);
#92156=CYLINDRICAL_SURFACE('',#109768,0.127000005450327);
#92157=CYLINDRICAL_SURFACE('',#109774,0.127);
#92158=CYLINDRICAL_SURFACE('',#109777,0.126999998753158);
#92159=CYLINDRICAL_SURFACE('',#109779,0.126999993595294);
#92160=CYLINDRICAL_SURFACE('',#109783,0.127);
#92161=CYLINDRICAL_SURFACE('',#109785,0.127);
#92162=CYLINDRICAL_SURFACE('',#109788,0.12700000030154);
#92163=CYLINDRICAL_SURFACE('',#109789,0.126999999706558);
#92164=CYLINDRICAL_SURFACE('',#109793,0.127);
#92165=CYLINDRICAL_SURFACE('',#109795,0.127);
#92166=CYLINDRICAL_SURFACE('',#109799,0.127000005438623);
#92167=CYLINDRICAL_SURFACE('',#109801,0.127000001278666);
#92168=CYLINDRICAL_SURFACE('',#109804,0.127);
#92169=CYLINDRICAL_SURFACE('',#109810,0.126999993616145);
#92170=CYLINDRICAL_SURFACE('',#109812,0.127000005453625);
#92171=CYLINDRICAL_SURFACE('',#109818,0.127000000000001);
#92172=CYLINDRICAL_SURFACE('',#109821,0.126999998751993);
#92173=CYLINDRICAL_SURFACE('',#109823,0.126999993594714);
#92174=CYLINDRICAL_SURFACE('',#109827,0.127000000000001);
#92175=CYLINDRICAL_SURFACE('',#109829,0.127000000000001);
#92176=CYLINDRICAL_SURFACE('',#109832,0.127000000299019);
#92177=CYLINDRICAL_SURFACE('',#109833,0.126999999706658);
#92178=CYLINDRICAL_SURFACE('',#109837,0.127);
#92179=CYLINDRICAL_SURFACE('',#109839,0.127);
#92180=CYLINDRICAL_SURFACE('',#109843,0.127000005436539);
#92181=CYLINDRICAL_SURFACE('',#109845,0.127000001278572);
#92182=CYLINDRICAL_SURFACE('',#109848,0.127);
#92183=CYLINDRICAL_SURFACE('',#109854,0.126999993618423);
#92184=CYLINDRICAL_SURFACE('',#109856,0.127000005451247);
#92185=CYLINDRICAL_SURFACE('',#109862,0.127);
#92186=CYLINDRICAL_SURFACE('',#109865,0.126999998752971);
#92187=CYLINDRICAL_SURFACE('',#109867,0.126999993593068);
#92188=CYLINDRICAL_SURFACE('',#109871,0.127);
#92189=CYLINDRICAL_SURFACE('',#109873,0.127);
#92190=CYLINDRICAL_SURFACE('',#109876,0.127000000302318);
#92191=CYLINDRICAL_SURFACE('',#109877,0.126999999707401);
#92192=CYLINDRICAL_SURFACE('',#109881,0.127);
#92193=CYLINDRICAL_SURFACE('',#109883,0.127);
#92194=CYLINDRICAL_SURFACE('',#109887,0.127000005436974);
#92195=CYLINDRICAL_SURFACE('',#109889,0.127000001280052);
#92196=CYLINDRICAL_SURFACE('',#109892,0.127);
#92197=CYLINDRICAL_SURFACE('',#109898,0.126999993617258);
#92198=CYLINDRICAL_SURFACE('',#109900,0.127000005450994);
#92199=CYLINDRICAL_SURFACE('',#109906,0.127);
#92200=CYLINDRICAL_SURFACE('',#109909,0.126999998752549);
#92201=CYLINDRICAL_SURFACE('',#109911,0.126999993591476);
#92202=CYLINDRICAL_SURFACE('',#109915,0.127);
#92203=CYLINDRICAL_SURFACE('',#109917,0.127);
#92204=CYLINDRICAL_SURFACE('',#109920,0.127000000302013);
#92205=CYLINDRICAL_SURFACE('',#109921,0.12699999970701);
#92206=CYLINDRICAL_SURFACE('',#109925,0.127);
#92207=CYLINDRICAL_SURFACE('',#109927,0.127);
#92208=CYLINDRICAL_SURFACE('',#109931,0.127000005437229);
#92209=CYLINDRICAL_SURFACE('',#109933,0.127000001279199);
#92210=CYLINDRICAL_SURFACE('',#109936,0.127);
#92211=CYLINDRICAL_SURFACE('',#109942,0.126999993615815);
#92212=CYLINDRICAL_SURFACE('',#109944,0.127000005452559);
#92213=CYLINDRICAL_SURFACE('',#109950,0.127000000000001);
#92214=CYLINDRICAL_SURFACE('',#109953,0.12699999875498);
#92215=CYLINDRICAL_SURFACE('',#109955,0.126999993591178);
#92216=CYLINDRICAL_SURFACE('',#109959,0.127000000000001);
#92217=CYLINDRICAL_SURFACE('',#109961,0.127000000000001);
#92218=CYLINDRICAL_SURFACE('',#109964,0.127000000300906);
#92219=CYLINDRICAL_SURFACE('',#109965,0.126999999707296);
#92220=CYLINDRICAL_SURFACE('',#109969,0.127);
#92221=CYLINDRICAL_SURFACE('',#109971,0.127);
#92222=CYLINDRICAL_SURFACE('',#109975,0.127000005438382);
#92223=CYLINDRICAL_SURFACE('',#109977,0.127000001277859);
#92224=CYLINDRICAL_SURFACE('',#109980,0.127);
#92225=CYLINDRICAL_SURFACE('',#109986,0.126999993613277);
#92226=CYLINDRICAL_SURFACE('',#109988,0.127000005457096);
#92227=CYLINDRICAL_SURFACE('',#109994,0.127000000000003);
#92228=CYLINDRICAL_SURFACE('',#109997,0.126999998755077);
#92229=CYLINDRICAL_SURFACE('',#109999,0.126999993597932);
#92230=CYLINDRICAL_SURFACE('',#110003,0.127000000000003);
#92231=CYLINDRICAL_SURFACE('',#110005,0.127000000000003);
#92232=CYLINDRICAL_SURFACE('',#110008,0.127000000302244);
#92233=CYLINDRICAL_SURFACE('',#110009,0.126999999705334);
#92234=CYLINDRICAL_SURFACE('',#110013,0.127);
#92235=CYLINDRICAL_SURFACE('',#110015,0.127);
#92236=CYLINDRICAL_SURFACE('',#110019,0.127000005437731);
#92237=CYLINDRICAL_SURFACE('',#110021,0.127000001278277);
#92238=CYLINDRICAL_SURFACE('',#110024,0.127);
#92239=CYLINDRICAL_SURFACE('',#110030,0.126999993613041);
#92240=CYLINDRICAL_SURFACE('',#110032,0.12700000545555);
#92241=CYLINDRICAL_SURFACE('',#110038,0.127000000000001);
#92242=CYLINDRICAL_SURFACE('',#110041,0.126999998754099);
#92243=CYLINDRICAL_SURFACE('',#110043,0.126999993597918);
#92244=CYLINDRICAL_SURFACE('',#110047,0.127000000000001);
#92245=CYLINDRICAL_SURFACE('',#110049,0.127000000000001);
#92246=CYLINDRICAL_SURFACE('',#110052,0.127000000302057);
#92247=CYLINDRICAL_SURFACE('',#110053,0.126999999706135);
#92248=CYLINDRICAL_SURFACE('',#110057,0.127);
#92249=CYLINDRICAL_SURFACE('',#110059,0.127);
#92250=CYLINDRICAL_SURFACE('',#110063,0.12700000543804);
#92251=CYLINDRICAL_SURFACE('',#110065,0.127000001278899);
#92252=CYLINDRICAL_SURFACE('',#110068,0.127);
#92253=CYLINDRICAL_SURFACE('',#110074,0.126999993615389);
#92254=CYLINDRICAL_SURFACE('',#110076,0.127000005454568);
#92255=CYLINDRICAL_SURFACE('',#110082,0.127);
#92256=CYLINDRICAL_SURFACE('',#110085,0.126999998752967);
#92257=CYLINDRICAL_SURFACE('',#110087,0.126999993594804);
#92258=CYLINDRICAL_SURFACE('',#110091,0.127);
#92259=CYLINDRICAL_SURFACE('',#110093,0.127);
#92260=CYLINDRICAL_SURFACE('',#110096,0.127000000301654);
#92261=CYLINDRICAL_SURFACE('',#110097,0.126999999706781);
#92262=CYLINDRICAL_SURFACE('',#110101,0.127);
#92263=CYLINDRICAL_SURFACE('',#110103,0.127);
#92264=CYLINDRICAL_SURFACE('',#110107,0.127000005439673);
#92265=CYLINDRICAL_SURFACE('',#110109,0.127000001277602);
#92266=CYLINDRICAL_SURFACE('',#110112,0.127);
#92267=CYLINDRICAL_SURFACE('',#110118,0.126999993615679);
#92268=CYLINDRICAL_SURFACE('',#110120,0.127000005451513);
#92269=CYLINDRICAL_SURFACE('',#110126,0.127000000000001);
#92270=CYLINDRICAL_SURFACE('',#110129,0.126999998752155);
#92271=CYLINDRICAL_SURFACE('',#110131,0.126999993594889);
#92272=CYLINDRICAL_SURFACE('',#110135,0.127000000000001);
#92273=CYLINDRICAL_SURFACE('',#110137,0.127000000000001);
#92274=CYLINDRICAL_SURFACE('',#110140,0.12700000030033);
#92275=CYLINDRICAL_SURFACE('',#110141,0.126999999705493);
#92276=CYLINDRICAL_SURFACE('',#110145,0.127);
#92277=CYLINDRICAL_SURFACE('',#110147,0.127);
#92278=CYLINDRICAL_SURFACE('',#110151,0.127000005438186);
#92279=CYLINDRICAL_SURFACE('',#110153,0.127000001279353);
#92280=CYLINDRICAL_SURFACE('',#110156,0.127);
#92281=CYLINDRICAL_SURFACE('',#110162,0.126999993616156);
#92282=CYLINDRICAL_SURFACE('',#110164,0.127000005452965);
#92283=CYLINDRICAL_SURFACE('',#110170,0.126999999999999);
#92284=CYLINDRICAL_SURFACE('',#110173,0.126999998753501);
#92285=CYLINDRICAL_SURFACE('',#110175,0.126999993594368);
#92286=CYLINDRICAL_SURFACE('',#110179,0.126999999999999);
#92287=CYLINDRICAL_SURFACE('',#110181,0.126999999999999);
#92288=CYLINDRICAL_SURFACE('',#110184,0.127000000302371);
#92289=CYLINDRICAL_SURFACE('',#110198,65.254);
#92290=CYLINDRICAL_SURFACE('',#110200,68.75);
#92291=CYLINDRICAL_SURFACE('',#110201,72.53);
#92292=CYLINDRICAL_SURFACE('',#110215,65.);
#92293=CYLINDRICAL_SURFACE('',#110217,65.254);
#92294=CYLINDRICAL_SURFACE('',#110259,2.54);
#92295=CYLINDRICAL_SURFACE('',#110261,2.54);
#92296=CYLINDRICAL_SURFACE('',#110266,72.53);
#92297=CYLINDRICAL_SURFACE('',#110269,8.4455);
#92298=CYLINDRICAL_SURFACE('',#110272,8.4455);
#92299=CYLINDRICAL_SURFACE('',#110275,8.4455);
#92300=CYLINDRICAL_SURFACE('',#110278,8.4455);
#92301=CYLINDRICAL_SURFACE('',#110281,80.);
#92302=CYLINDRICAL_SURFACE('',#110292,25.);
#92303=CYLINDRICAL_SURFACE('',#110297,25.);
#92304=CYLINDRICAL_SURFACE('',#110305,25.);
#92305=CYLINDRICAL_SURFACE('',#110309,25.);
#92306=CYLINDRICAL_SURFACE('',#110314,24.492);
#92307=CYLINDRICAL_SURFACE('',#110318,24.492);
#92308=CYLINDRICAL_SURFACE('',#110322,24.492);
#92309=CYLINDRICAL_SURFACE('',#110326,24.492);
#92310=CYLINDRICAL_SURFACE('',#110336,81.2699999999993);
#92311=CYLINDRICAL_SURFACE('',#110338,80.);
#92312=CYLINDRICAL_SURFACE('',#110348,80.);
#92313=CYLINDRICAL_SURFACE('',#110353,80.);
#92314=CYLINDRICAL_SURFACE('',#110358,80.);
#92315=CYLINDRICAL_SURFACE('',#110396,2.54);
#92316=CYLINDRICAL_SURFACE('',#110399,2.54);
#92317=CYLINDRICAL_SURFACE('',#110402,2.54);
#92318=CYLINDRICAL_SURFACE('',#110404,2.54);
#92319=CYLINDRICAL_SURFACE('',#110406,2.54);
#92320=CYLINDRICAL_SURFACE('',#110408,2.54);
#92321=CYLINDRICAL_SURFACE('',#110412,1.905);
#92322=CYLINDRICAL_SURFACE('',#110419,1.905);
#92323=CYLINDRICAL_SURFACE('',#110421,1.905);
#92324=CYLINDRICAL_SURFACE('',#110424,1.905);
#92325=CYLINDRICAL_SURFACE('',#110428,1.905);
#92326=CYLINDRICAL_SURFACE('',#110430,1.905);
#92327=CYLINDRICAL_SURFACE('',#110433,1.905);
#92328=CYLINDRICAL_SURFACE('',#110438,1.905);
#92329=CYLINDRICAL_SURFACE('',#110440,1.905);
#92330=CYLINDRICAL_SURFACE('',#110443,1.905);
#92331=CYLINDRICAL_SURFACE('',#110447,1.905);
#92332=CYLINDRICAL_SURFACE('',#110449,1.27);
#92333=CYLINDRICAL_SURFACE('',#110453,1.27);
#92334=CYLINDRICAL_SURFACE('',#110454,1.27);
#92335=CYLINDRICAL_SURFACE('',#110455,1.27);
#92336=CYLINDRICAL_SURFACE('',#110456,1.27);
#92337=CYLINDRICAL_SURFACE('',#110457,1.27);
#92338=CYLINDRICAL_SURFACE('',#110458,1.27);
#92339=CYLINDRICAL_SURFACE('',#110462,1.27);
#92340=CYLINDRICAL_SURFACE('',#110478,1.27);
#92341=CYLINDRICAL_SURFACE('',#110481,1.27);
#92342=CYLINDRICAL_SURFACE('',#110504,2.54);
#92343=CYLINDRICAL_SURFACE('',#110507,2.54);
#92344=CYLINDRICAL_SURFACE('',#110523,66.0360441972308);
#92345=CYLINDRICAL_SURFACE('',#110524,1.27);
#92346=CYLINDRICAL_SURFACE('',#110527,1.905);
#92347=CYLINDRICAL_SURFACE('',#110541,1.27);
#92348=CYLINDRICAL_SURFACE('',#110542,66.0995441972308);
#92349=CYLINDRICAL_SURFACE('',#110544,66.4805441972308);
#92350=CYLINDRICAL_SURFACE('',#110570,56.875);
#92351=CYLINDRICAL_SURFACE('',#110575,51.27);
#92352=CYLINDRICAL_SURFACE('',#110577,50.);
#92353=CYLINDRICAL_SURFACE('',#110579,65.);
#92354=CYLINDRICAL_SURFACE('',#110587,4.7227367061318);
#92355=CYLINDRICAL_SURFACE('',#110589,4.7227367061318);
#92356=CYLINDRICAL_SURFACE('',#110590,4.7227367061318);
#92357=CYLINDRICAL_SURFACE('',#110591,4.7227367061318);
#92358=CYLINDRICAL_SURFACE('',#110592,4.7227367061318);
#92359=CYLINDRICAL_SURFACE('',#110593,4.7227367061318);
#92360=CYLINDRICAL_SURFACE('',#110594,4.74980000000001);
#92361=CYLINDRICAL_SURFACE('',#110596,4.74980000000001);
#92362=CYLINDRICAL_SURFACE('',#110598,4.74980000000001);
#92363=CYLINDRICAL_SURFACE('',#110599,4.74980000000001);
#92364=CYLINDRICAL_SURFACE('',#110600,4.74980000000001);
#92365=CYLINDRICAL_SURFACE('',#110601,4.74980000000001);
#92366=CYLINDRICAL_SURFACE('',#110602,4.74980000000001);
#92367=CYLINDRICAL_SURFACE('',#110603,4.74980000000001);
#92368=CYLINDRICAL_SURFACE('',#110616,4.74980000000001);
#92369=CYLINDRICAL_SURFACE('',#110638,4.7227367061318);
#92370=CYLINDRICAL_SURFACE('',#110639,4.72273670613179);
#92371=CYLINDRICAL_SURFACE('',#110641,4.72273670613179);
#92372=CYLINDRICAL_SURFACE('',#110642,4.72273670613179);
#92373=CYLINDRICAL_SURFACE('',#110643,4.72273670613179);
#92374=CYLINDRICAL_SURFACE('',#110644,4.72273670613179);
#92375=CYLINDRICAL_SURFACE('',#110645,4.72273670613179);
#92376=CYLINDRICAL_SURFACE('',#110646,4.74980000000001);
#92377=CYLINDRICAL_SURFACE('',#110648,4.74980000000001);
#92378=CYLINDRICAL_SURFACE('',#110650,4.74980000000001);
#92379=CYLINDRICAL_SURFACE('',#110651,4.74980000000001);
#92380=CYLINDRICAL_SURFACE('',#110652,4.74980000000001);
#92381=CYLINDRICAL_SURFACE('',#110653,4.74980000000001);
#92382=CYLINDRICAL_SURFACE('',#110654,4.74980000000001);
#92383=CYLINDRICAL_SURFACE('',#110655,4.74980000000001);
#92384=CYLINDRICAL_SURFACE('',#110668,4.74980000000001);
#92385=CYLINDRICAL_SURFACE('',#110690,4.72273670613179);
#92386=CYLINDRICAL_SURFACE('',#110705,50.);
#92387=CYLINDRICAL_SURFACE('',#110706,4.7625);
#92388=CYLINDRICAL_SURFACE('',#110707,4.7625);
#92389=CYLINDRICAL_SURFACE('',#110708,40.);
#92390=CYLINDRICAL_SURFACE('',#110711,65.0000000000002);
#92391=CYLINDRICAL_SURFACE('',#110714,56.875);
#92392=CYLINDRICAL_SURFACE('',#110722,76.4577478255888);
#92393=CYLINDRICAL_SURFACE('',#110724,66.9885441972308);
#92394=CYLINDRICAL_SURFACE('',#110727,70.625);
#92395=CYLINDRICAL_SURFACE('',#110730,76.5847478255888);
#92396=CYLINDRICAL_SURFACE('',#110733,8.4455);
#92397=CYLINDRICAL_SURFACE('',#110736,8.4455);
#92398=CYLINDRICAL_SURFACE('',#110739,8.4455);
#92399=CYLINDRICAL_SURFACE('',#110742,8.4455);
#92400=CYLINDRICAL_SURFACE('',#110745,7.9375);
#92401=CYLINDRICAL_SURFACE('',#110748,7.9375);
#92402=CYLINDRICAL_SURFACE('',#110751,7.9375);
#92403=CYLINDRICAL_SURFACE('',#110754,7.9375);
#92404=CYLINDRICAL_SURFACE('',#110757,24.492);
#92405=CYLINDRICAL_SURFACE('',#110761,24.492);
#92406=CYLINDRICAL_SURFACE('',#110765,24.492);
#92407=CYLINDRICAL_SURFACE('',#110769,24.492);
#92408=CYLINDRICAL_SURFACE('',#110787,25.);
#92409=CYLINDRICAL_SURFACE('',#110790,25.);
#92410=CYLINDRICAL_SURFACE('',#110793,25.);
#92411=CYLINDRICAL_SURFACE('',#110796,25.);
#92412=CYLINDRICAL_SURFACE('',#110802,0.761999999999999);
#92413=CYLINDRICAL_SURFACE('',#110804,0.762);
#92414=CYLINDRICAL_SURFACE('',#110810,0.762);
#92415=CYLINDRICAL_SURFACE('',#110812,0.762);
#92416=CYLINDRICAL_SURFACE('',#110816,66.9885441972308);
#92417=CYLINDRICAL_SURFACE('',#110825,73.6560441972308);
#92418=CYLINDRICAL_SURFACE('',#110831,73.6560441972308);
#92680=ADVANCED_FACE('',(#7707),#5535,.F.);
#92681=ADVANCED_FACE('',(#7708),#90343,.T.);
#92682=ADVANCED_FACE('',(#7709),#50,.T.);
#92683=ADVANCED_FACE('',(#7710),#90344,.T.);
#92684=ADVANCED_FACE('',(#7711),#51,.T.);
#92685=ADVANCED_FACE('',(#7712),#52,.T.);
#92686=ADVANCED_FACE('',(#7713,#6349),#45,.T.);
#92687=ADVANCED_FACE('',(#7714),#5536,.T.);
#92688=ADVANCED_FACE('',(#7715),#53,.T.);
#92689=ADVANCED_FACE('',(#7716),#5537,.T.);
#92690=ADVANCED_FACE('',(#7717),#90345,.F.);
#92691=ADVANCED_FACE('',(#7718,#6350),#6478,.T.);
#92692=ADVANCED_FACE('',(#7719),#6479,.T.);
#92693=ADVANCED_FACE('',(#7720),#54,.T.);
#92694=ADVANCED_FACE('',(#7721),#55,.T.);
#92695=ADVANCED_FACE('',(#7722),#56,.T.);
#92696=ADVANCED_FACE('',(#7723),#57,.T.);
#92697=ADVANCED_FACE('',(#7724),#58,.T.);
#92698=ADVANCED_FACE('',(#7725),#6480,.T.);
#92699=ADVANCED_FACE('',(#7726,#6351),#6481,.T.);
#92700=ADVANCED_FACE('',(#7727),#59,.T.);
#92701=ADVANCED_FACE('',(#7728),#60,.T.);
#92702=ADVANCED_FACE('',(#7729),#61,.T.);
#92703=ADVANCED_FACE('',(#7730),#62,.T.);
#92704=ADVANCED_FACE('',(#7731),#63,.T.);
#92705=ADVANCED_FACE('',(#7732),#6482,.T.);
#92706=ADVANCED_FACE('',(#7733),#6483,.T.);
#92707=ADVANCED_FACE('',(#7734),#6484,.T.);
#92708=ADVANCED_FACE('',(#7735),#6485,.T.);
#92709=ADVANCED_FACE('',(#7736),#6486,.T.);
#92710=ADVANCED_FACE('',(#7737),#6487,.T.);
#92711=ADVANCED_FACE('',(#7738),#90346,.T.);
#92712=ADVANCED_FACE('',(#7739),#90347,.T.);
#92713=ADVANCED_FACE('',(#7740),#90348,.T.);
#92714=ADVANCED_FACE('',(#7741),#90349,.T.);
#92715=ADVANCED_FACE('',(#7742),#90350,.T.);
#92716=ADVANCED_FACE('',(#7743),#90351,.F.);
#92717=ADVANCED_FACE('',(#7744),#90352,.T.);
#92718=ADVANCED_FACE('',(#7745,#6352),#6488,.F.);
#92719=ADVANCED_FACE('',(#7746,#6353),#6489,.T.);
#92720=ADVANCED_FACE('',(#7747),#90353,.F.);
#92721=ADVANCED_FACE('',(#7748),#90354,.T.);
#92722=ADVANCED_FACE('',(#7749,#6354),#6490,.F.);
#92723=ADVANCED_FACE('',(#7750,#6355),#6491,.T.);
#92724=ADVANCED_FACE('',(#7751),#90355,.F.);
#92725=ADVANCED_FACE('',(#7752),#90356,.T.);
#92726=ADVANCED_FACE('',(#7753,#6356),#6492,.F.);
#92727=ADVANCED_FACE('',(#7754,#6357),#6493,.T.);
#92728=ADVANCED_FACE('',(#7755),#90357,.F.);
#92729=ADVANCED_FACE('',(#7756),#90358,.T.);
#92730=ADVANCED_FACE('',(#7757,#6358),#6494,.F.);
#92731=ADVANCED_FACE('',(#7758,#6359),#6495,.T.);
#92732=ADVANCED_FACE('',(#7759),#5538,.T.);
#92733=ADVANCED_FACE('',(#7760),#5539,.T.);
#92734=ADVANCED_FACE('',(#7761),#90359,.T.);
#92735=ADVANCED_FACE('',(#7762),#90360,.F.);
#92736=ADVANCED_FACE('',(#7763,#6360),#6496,.F.);
#92737=ADVANCED_FACE('',(#7764,#6361),#6497,.T.);
#92738=ADVANCED_FACE('',(#7765),#5540,.T.);
#92739=ADVANCED_FACE('',(#7766),#5541,.T.);
#92740=ADVANCED_FACE('',(#7767),#90361,.T.);
#92741=ADVANCED_FACE('',(#7768),#90362,.F.);
#92742=ADVANCED_FACE('',(#7769,#6362),#6498,.F.);
#92743=ADVANCED_FACE('',(#7770,#6363),#6499,.T.);
#92744=ADVANCED_FACE('',(#7771),#90363,.F.);
#92745=ADVANCED_FACE('',(#7772),#90364,.T.);
#92746=ADVANCED_FACE('',(#7773,#6364),#6500,.F.);
#92747=ADVANCED_FACE('',(#7774,#6365),#6501,.T.);
#92748=ADVANCED_FACE('',(#7775),#5542,.F.);
#92749=ADVANCED_FACE('',(#7776),#5543,.F.);
#92750=ADVANCED_FACE('',(#7777),#5544,.F.);
#92751=ADVANCED_FACE('',(#7778),#5545,.F.);
#92752=ADVANCED_FACE('',(#7779),#5546,.T.);
#92753=ADVANCED_FACE('',(#7780),#5547,.T.);
#92754=ADVANCED_FACE('',(#7781),#5548,.T.);
#92755=ADVANCED_FACE('',(#7782),#5549,.T.);
#92756=ADVANCED_FACE('',(#7783),#90365,.T.);
#92757=ADVANCED_FACE('',(#7784),#64,.T.);
#92758=ADVANCED_FACE('',(#7785),#65,.F.);
#92759=ADVANCED_FACE('',(#7786),#66,.T.);
#92760=ADVANCED_FACE('',(#7787),#67,.F.);
#92761=ADVANCED_FACE('',(#7788),#90366,.F.);
#92762=ADVANCED_FACE('',(#7789),#6502,.F.);
#92763=ADVANCED_FACE('',(#7790),#68,.F.);
#92764=ADVANCED_FACE('',(#7791),#6503,.F.);
#92765=ADVANCED_FACE('',(#7792),#69,.T.);
#92766=ADVANCED_FACE('',(#7793),#6504,.F.);
#92767=ADVANCED_FACE('',(#7794),#5550,.F.);
#92768=ADVANCED_FACE('',(#7795),#5551,.F.);
#92769=ADVANCED_FACE('',(#7796),#5552,.T.);
#92770=ADVANCED_FACE('',(#7797),#5553,.T.);
#92771=ADVANCED_FACE('',(#7798),#6505,.F.);
#92772=ADVANCED_FACE('',(#7799),#70,.F.);
#92773=ADVANCED_FACE('',(#7800),#6506,.F.);
#92774=ADVANCED_FACE('',(#7801),#71,.T.);
#92775=ADVANCED_FACE('',(#7802),#6507,.F.);
#92776=ADVANCED_FACE('',(#7803),#5554,.F.);
#92777=ADVANCED_FACE('',(#7804),#5555,.F.);
#92778=ADVANCED_FACE('',(#7805),#5556,.T.);
#92779=ADVANCED_FACE('',(#7806),#5557,.T.);
#92780=ADVANCED_FACE('',(#7807),#6508,.F.);
#92781=ADVANCED_FACE('',(#7808),#72,.F.);
#92782=ADVANCED_FACE('',(#7809),#6509,.F.);
#92783=ADVANCED_FACE('',(#7810),#73,.T.);
#92784=ADVANCED_FACE('',(#7811),#6510,.F.);
#92785=ADVANCED_FACE('',(#7812),#5558,.F.);
#92786=ADVANCED_FACE('',(#7813),#5559,.F.);
#92787=ADVANCED_FACE('',(#7814),#5560,.T.);
#92788=ADVANCED_FACE('',(#7815),#5561,.T.);
#92789=ADVANCED_FACE('',(#7816),#6511,.F.);
#92790=ADVANCED_FACE('',(#7817),#74,.F.);
#92791=ADVANCED_FACE('',(#7818),#6512,.F.);
#92792=ADVANCED_FACE('',(#7819),#75,.T.);
#92793=ADVANCED_FACE('',(#7820),#6513,.F.);
#92794=ADVANCED_FACE('',(#7821),#5562,.F.);
#92795=ADVANCED_FACE('',(#7822),#5563,.F.);
#92796=ADVANCED_FACE('',(#7823),#5564,.T.);
#92797=ADVANCED_FACE('',(#7824),#5565,.T.);
#92798=ADVANCED_FACE('',(#7825),#6514,.F.);
#92799=ADVANCED_FACE('',(#7826),#76,.F.);
#92800=ADVANCED_FACE('',(#7827),#6515,.F.);
#92801=ADVANCED_FACE('',(#7828),#77,.T.);
#92802=ADVANCED_FACE('',(#7829),#6516,.F.);
#92803=ADVANCED_FACE('',(#7830),#5566,.F.);
#92804=ADVANCED_FACE('',(#7831),#5567,.F.);
#92805=ADVANCED_FACE('',(#7832),#5568,.T.);
#92806=ADVANCED_FACE('',(#7833),#5569,.T.);
#92807=ADVANCED_FACE('',(#7834),#6517,.F.);
#92808=ADVANCED_FACE('',(#7835),#78,.F.);
#92809=ADVANCED_FACE('',(#7836),#6518,.F.);
#92810=ADVANCED_FACE('',(#7837),#79,.T.);
#92811=ADVANCED_FACE('',(#7838),#6519,.F.);
#92812=ADVANCED_FACE('',(#7839),#5570,.F.);
#92813=ADVANCED_FACE('',(#7840),#5571,.F.);
#92814=ADVANCED_FACE('',(#7841),#5572,.T.);
#92815=ADVANCED_FACE('',(#7842),#5573,.T.);
#92816=ADVANCED_FACE('',(#7843),#6520,.F.);
#92817=ADVANCED_FACE('',(#7844),#80,.F.);
#92818=ADVANCED_FACE('',(#7845),#6521,.F.);
#92819=ADVANCED_FACE('',(#7846),#81,.T.);
#92820=ADVANCED_FACE('',(#7847),#6522,.F.);
#92821=ADVANCED_FACE('',(#7848),#5574,.F.);
#92822=ADVANCED_FACE('',(#7849),#5575,.F.);
#92823=ADVANCED_FACE('',(#7850),#5576,.T.);
#92824=ADVANCED_FACE('',(#7851),#5577,.T.);
#92825=ADVANCED_FACE('',(#7852),#6523,.F.);
#92826=ADVANCED_FACE('',(#7853),#82,.F.);
#92827=ADVANCED_FACE('',(#7854),#6524,.F.);
#92828=ADVANCED_FACE('',(#7855),#83,.T.);
#92829=ADVANCED_FACE('',(#7856),#6525,.F.);
#92830=ADVANCED_FACE('',(#7857),#5578,.F.);
#92831=ADVANCED_FACE('',(#7858),#5579,.F.);
#92832=ADVANCED_FACE('',(#7859),#5580,.T.);
#92833=ADVANCED_FACE('',(#7860),#5581,.T.);
#92834=ADVANCED_FACE('',(#7861),#6526,.F.);
#92835=ADVANCED_FACE('',(#7862),#84,.F.);
#92836=ADVANCED_FACE('',(#7863),#6527,.F.);
#92837=ADVANCED_FACE('',(#7864),#85,.T.);
#92838=ADVANCED_FACE('',(#7865),#6528,.F.);
#92839=ADVANCED_FACE('',(#7866),#5582,.F.);
#92840=ADVANCED_FACE('',(#7867),#5583,.F.);
#92841=ADVANCED_FACE('',(#7868),#5584,.T.);
#92842=ADVANCED_FACE('',(#7869),#5585,.T.);
#92843=ADVANCED_FACE('',(#7870),#6529,.F.);
#92844=ADVANCED_FACE('',(#7871),#86,.F.);
#92845=ADVANCED_FACE('',(#7872),#6530,.F.);
#92846=ADVANCED_FACE('',(#7873),#87,.T.);
#92847=ADVANCED_FACE('',(#7874),#6531,.F.);
#92848=ADVANCED_FACE('',(#7875),#5586,.F.);
#92849=ADVANCED_FACE('',(#7876),#5587,.F.);
#92850=ADVANCED_FACE('',(#7877),#5588,.T.);
#92851=ADVANCED_FACE('',(#7878),#5589,.T.);
#92852=ADVANCED_FACE('',(#7879),#6532,.F.);
#92853=ADVANCED_FACE('',(#7880),#88,.F.);
#92854=ADVANCED_FACE('',(#7881),#6533,.F.);
#92855=ADVANCED_FACE('',(#7882),#89,.T.);
#92856=ADVANCED_FACE('',(#7883),#6534,.F.);
#92857=ADVANCED_FACE('',(#7884),#5590,.F.);
#92858=ADVANCED_FACE('',(#7885),#5591,.F.);
#92859=ADVANCED_FACE('',(#7886),#5592,.T.);
#92860=ADVANCED_FACE('',(#7887),#5593,.T.);
#92861=ADVANCED_FACE('',(#7888),#6535,.F.);
#92862=ADVANCED_FACE('',(#7889),#90,.F.);
#92863=ADVANCED_FACE('',(#7890),#6536,.F.);
#92864=ADVANCED_FACE('',(#7891),#91,.T.);
#92865=ADVANCED_FACE('',(#7892),#6537,.F.);
#92866=ADVANCED_FACE('',(#7893),#5594,.F.);
#92867=ADVANCED_FACE('',(#7894),#5595,.F.);
#92868=ADVANCED_FACE('',(#7895),#5596,.T.);
#92869=ADVANCED_FACE('',(#7896),#5597,.T.);
#92870=ADVANCED_FACE('',(#7897),#6538,.F.);
#92871=ADVANCED_FACE('',(#7898),#92,.F.);
#92872=ADVANCED_FACE('',(#7899),#6539,.F.);
#92873=ADVANCED_FACE('',(#7900),#93,.T.);
#92874=ADVANCED_FACE('',(#7901),#6540,.F.);
#92875=ADVANCED_FACE('',(#7902),#5598,.F.);
#92876=ADVANCED_FACE('',(#7903),#5599,.F.);
#92877=ADVANCED_FACE('',(#7904),#5600,.T.);
#92878=ADVANCED_FACE('',(#7905),#5601,.T.);
#92879=ADVANCED_FACE('',(#7906),#6541,.F.);
#92880=ADVANCED_FACE('',(#7907),#94,.F.);
#92881=ADVANCED_FACE('',(#7908),#6542,.F.);
#92882=ADVANCED_FACE('',(#7909),#95,.T.);
#92883=ADVANCED_FACE('',(#7910),#6543,.F.);
#92884=ADVANCED_FACE('',(#7911),#5602,.F.);
#92885=ADVANCED_FACE('',(#7912),#5603,.F.);
#92886=ADVANCED_FACE('',(#7913),#5604,.T.);
#92887=ADVANCED_FACE('',(#7914),#5605,.T.);
#92888=ADVANCED_FACE('',(#7915),#6544,.F.);
#92889=ADVANCED_FACE('',(#7916),#96,.F.);
#92890=ADVANCED_FACE('',(#7917),#6545,.F.);
#92891=ADVANCED_FACE('',(#7918),#97,.T.);
#92892=ADVANCED_FACE('',(#7919),#6546,.F.);
#92893=ADVANCED_FACE('',(#7920),#5606,.F.);
#92894=ADVANCED_FACE('',(#7921),#5607,.F.);
#92895=ADVANCED_FACE('',(#7922),#5608,.T.);
#92896=ADVANCED_FACE('',(#7923),#5609,.T.);
#92897=ADVANCED_FACE('',(#7924),#6547,.F.);
#92898=ADVANCED_FACE('',(#7925),#98,.F.);
#92899=ADVANCED_FACE('',(#7926),#6548,.F.);
#92900=ADVANCED_FACE('',(#7927),#99,.T.);
#92901=ADVANCED_FACE('',(#7928),#6549,.F.);
#92902=ADVANCED_FACE('',(#7929),#5610,.F.);
#92903=ADVANCED_FACE('',(#7930),#5611,.F.);
#92904=ADVANCED_FACE('',(#7931),#5612,.T.);
#92905=ADVANCED_FACE('',(#7932),#5613,.T.);
#92906=ADVANCED_FACE('',(#7933),#6550,.F.);
#92907=ADVANCED_FACE('',(#7934),#100,.F.);
#92908=ADVANCED_FACE('',(#7935),#6551,.F.);
#92909=ADVANCED_FACE('',(#7936),#101,.T.);
#92910=ADVANCED_FACE('',(#7937),#6552,.F.);
#92911=ADVANCED_FACE('',(#7938),#5614,.F.);
#92912=ADVANCED_FACE('',(#7939),#5615,.F.);
#92913=ADVANCED_FACE('',(#7940),#5616,.T.);
#92914=ADVANCED_FACE('',(#7941),#5617,.T.);
#92915=ADVANCED_FACE('',(#7942),#6553,.F.);
#92916=ADVANCED_FACE('',(#7943),#102,.F.);
#92917=ADVANCED_FACE('',(#7944),#6554,.F.);
#92918=ADVANCED_FACE('',(#7945),#103,.T.);
#92919=ADVANCED_FACE('',(#7946),#6555,.F.);
#92920=ADVANCED_FACE('',(#7947),#5618,.F.);
#92921=ADVANCED_FACE('',(#7948),#5619,.F.);
#92922=ADVANCED_FACE('',(#7949),#5620,.T.);
#92923=ADVANCED_FACE('',(#7950),#5621,.T.);
#92924=ADVANCED_FACE('',(#7951),#6556,.F.);
#92925=ADVANCED_FACE('',(#7952),#104,.F.);
#92926=ADVANCED_FACE('',(#7953),#6557,.F.);
#92927=ADVANCED_FACE('',(#7954),#105,.T.);
#92928=ADVANCED_FACE('',(#7955),#6558,.F.);
#92929=ADVANCED_FACE('',(#7956),#5622,.F.);
#92930=ADVANCED_FACE('',(#7957),#5623,.F.);
#92931=ADVANCED_FACE('',(#7958),#5624,.T.);
#92932=ADVANCED_FACE('',(#7959),#5625,.T.);
#92933=ADVANCED_FACE('',(#7960),#6559,.F.);
#92934=ADVANCED_FACE('',(#7961),#106,.F.);
#92935=ADVANCED_FACE('',(#7962),#6560,.F.);
#92936=ADVANCED_FACE('',(#7963),#107,.T.);
#92937=ADVANCED_FACE('',(#7964),#6561,.F.);
#92938=ADVANCED_FACE('',(#7965),#5626,.F.);
#92939=ADVANCED_FACE('',(#7966),#5627,.F.);
#92940=ADVANCED_FACE('',(#7967),#5628,.T.);
#92941=ADVANCED_FACE('',(#7968),#5629,.T.);
#92942=ADVANCED_FACE('',(#7969),#6562,.F.);
#92943=ADVANCED_FACE('',(#7970),#108,.F.);
#92944=ADVANCED_FACE('',(#7971),#6563,.F.);
#92945=ADVANCED_FACE('',(#7972),#109,.T.);
#92946=ADVANCED_FACE('',(#7973),#6564,.F.);
#92947=ADVANCED_FACE('',(#7974),#5630,.F.);
#92948=ADVANCED_FACE('',(#7975),#5631,.F.);
#92949=ADVANCED_FACE('',(#7976),#5632,.T.);
#92950=ADVANCED_FACE('',(#7977),#5633,.T.);
#92951=ADVANCED_FACE('',(#7978),#6565,.F.);
#92952=ADVANCED_FACE('',(#7979),#110,.F.);
#92953=ADVANCED_FACE('',(#7980),#6566,.F.);
#92954=ADVANCED_FACE('',(#7981),#111,.T.);
#92955=ADVANCED_FACE('',(#7982),#6567,.F.);
#92956=ADVANCED_FACE('',(#7983),#5634,.F.);
#92957=ADVANCED_FACE('',(#7984),#5635,.F.);
#92958=ADVANCED_FACE('',(#7985),#5636,.T.);
#92959=ADVANCED_FACE('',(#7986),#5637,.T.);
#92960=ADVANCED_FACE('',(#7987),#6568,.F.);
#92961=ADVANCED_FACE('',(#7988),#112,.F.);
#92962=ADVANCED_FACE('',(#7989),#6569,.F.);
#92963=ADVANCED_FACE('',(#7990),#113,.T.);
#92964=ADVANCED_FACE('',(#7991),#6570,.F.);
#92965=ADVANCED_FACE('',(#7992),#5638,.F.);
#92966=ADVANCED_FACE('',(#7993),#5639,.F.);
#92967=ADVANCED_FACE('',(#7994),#5640,.T.);
#92968=ADVANCED_FACE('',(#7995),#5641,.T.);
#92969=ADVANCED_FACE('',(#7996),#6571,.F.);
#92970=ADVANCED_FACE('',(#7997),#114,.F.);
#92971=ADVANCED_FACE('',(#7998),#6572,.F.);
#92972=ADVANCED_FACE('',(#7999),#115,.T.);
#92973=ADVANCED_FACE('',(#8000),#6573,.F.);
#92974=ADVANCED_FACE('',(#8001),#5642,.F.);
#92975=ADVANCED_FACE('',(#8002),#5643,.F.);
#92976=ADVANCED_FACE('',(#8003),#5644,.T.);
#92977=ADVANCED_FACE('',(#8004),#5645,.T.);
#92978=ADVANCED_FACE('',(#8005),#6574,.F.);
#92979=ADVANCED_FACE('',(#8006),#116,.F.);
#92980=ADVANCED_FACE('',(#8007),#6575,.F.);
#92981=ADVANCED_FACE('',(#8008),#117,.T.);
#92982=ADVANCED_FACE('',(#8009),#6576,.F.);
#92983=ADVANCED_FACE('',(#8010),#5646,.F.);
#92984=ADVANCED_FACE('',(#8011),#5647,.F.);
#92985=ADVANCED_FACE('',(#8012),#5648,.T.);
#92986=ADVANCED_FACE('',(#8013),#5649,.T.);
#92987=ADVANCED_FACE('',(#8014),#6577,.F.);
#92988=ADVANCED_FACE('',(#8015),#118,.F.);
#92989=ADVANCED_FACE('',(#8016),#6578,.F.);
#92990=ADVANCED_FACE('',(#8017),#119,.T.);
#92991=ADVANCED_FACE('',(#8018),#6579,.F.);
#92992=ADVANCED_FACE('',(#8019),#5650,.F.);
#92993=ADVANCED_FACE('',(#8020),#5651,.F.);
#92994=ADVANCED_FACE('',(#8021),#5652,.T.);
#92995=ADVANCED_FACE('',(#8022),#5653,.T.);
#92996=ADVANCED_FACE('',(#8023),#6580,.F.);
#92997=ADVANCED_FACE('',(#8024),#120,.F.);
#92998=ADVANCED_FACE('',(#8025),#6581,.F.);
#92999=ADVANCED_FACE('',(#8026),#121,.T.);
#93000=ADVANCED_FACE('',(#8027),#6582,.F.);
#93001=ADVANCED_FACE('',(#8028),#5654,.F.);
#93002=ADVANCED_FACE('',(#8029),#5655,.F.);
#93003=ADVANCED_FACE('',(#8030),#5656,.T.);
#93004=ADVANCED_FACE('',(#8031),#5657,.T.);
#93005=ADVANCED_FACE('',(#8032),#6583,.F.);
#93006=ADVANCED_FACE('',(#8033),#122,.F.);
#93007=ADVANCED_FACE('',(#8034),#6584,.F.);
#93008=ADVANCED_FACE('',(#8035),#123,.T.);
#93009=ADVANCED_FACE('',(#8036),#6585,.F.);
#93010=ADVANCED_FACE('',(#8037),#5658,.F.);
#93011=ADVANCED_FACE('',(#8038),#5659,.F.);
#93012=ADVANCED_FACE('',(#8039),#5660,.T.);
#93013=ADVANCED_FACE('',(#8040),#5661,.T.);
#93014=ADVANCED_FACE('',(#8041),#6586,.F.);
#93015=ADVANCED_FACE('',(#8042),#124,.F.);
#93016=ADVANCED_FACE('',(#8043),#6587,.F.);
#93017=ADVANCED_FACE('',(#8044),#125,.T.);
#93018=ADVANCED_FACE('',(#8045),#6588,.F.);
#93019=ADVANCED_FACE('',(#8046),#5662,.F.);
#93020=ADVANCED_FACE('',(#8047),#5663,.F.);
#93021=ADVANCED_FACE('',(#8048),#5664,.T.);
#93022=ADVANCED_FACE('',(#8049),#5665,.T.);
#93023=ADVANCED_FACE('',(#8050),#6589,.F.);
#93024=ADVANCED_FACE('',(#8051),#126,.F.);
#93025=ADVANCED_FACE('',(#8052),#6590,.F.);
#93026=ADVANCED_FACE('',(#8053),#127,.T.);
#93027=ADVANCED_FACE('',(#8054),#6591,.F.);
#93028=ADVANCED_FACE('',(#8055),#5666,.F.);
#93029=ADVANCED_FACE('',(#8056),#5667,.F.);
#93030=ADVANCED_FACE('',(#8057),#5668,.T.);
#93031=ADVANCED_FACE('',(#8058),#5669,.T.);
#93032=ADVANCED_FACE('',(#8059),#6592,.F.);
#93033=ADVANCED_FACE('',(#8060),#128,.F.);
#93034=ADVANCED_FACE('',(#8061),#6593,.F.);
#93035=ADVANCED_FACE('',(#8062),#129,.T.);
#93036=ADVANCED_FACE('',(#8063),#6594,.F.);
#93037=ADVANCED_FACE('',(#8064),#5670,.F.);
#93038=ADVANCED_FACE('',(#8065),#5671,.F.);
#93039=ADVANCED_FACE('',(#8066),#5672,.T.);
#93040=ADVANCED_FACE('',(#8067),#5673,.T.);
#93041=ADVANCED_FACE('',(#8068),#6595,.F.);
#93042=ADVANCED_FACE('',(#8069),#130,.F.);
#93043=ADVANCED_FACE('',(#8070),#6596,.F.);
#93044=ADVANCED_FACE('',(#8071),#131,.T.);
#93045=ADVANCED_FACE('',(#8072),#6597,.F.);
#93046=ADVANCED_FACE('',(#8073),#5674,.F.);
#93047=ADVANCED_FACE('',(#8074),#5675,.F.);
#93048=ADVANCED_FACE('',(#8075),#5676,.T.);
#93049=ADVANCED_FACE('',(#8076),#5677,.T.);
#93050=ADVANCED_FACE('',(#8077),#6598,.F.);
#93051=ADVANCED_FACE('',(#8078),#132,.F.);
#93052=ADVANCED_FACE('',(#8079),#6599,.F.);
#93053=ADVANCED_FACE('',(#8080),#133,.T.);
#93054=ADVANCED_FACE('',(#8081),#6600,.F.);
#93055=ADVANCED_FACE('',(#8082),#5678,.F.);
#93056=ADVANCED_FACE('',(#8083),#5679,.F.);
#93057=ADVANCED_FACE('',(#8084),#5680,.T.);
#93058=ADVANCED_FACE('',(#8085),#5681,.T.);
#93059=ADVANCED_FACE('',(#8086),#6601,.F.);
#93060=ADVANCED_FACE('',(#8087),#134,.F.);
#93061=ADVANCED_FACE('',(#8088),#6602,.F.);
#93062=ADVANCED_FACE('',(#8089),#135,.T.);
#93063=ADVANCED_FACE('',(#8090),#6603,.F.);
#93064=ADVANCED_FACE('',(#8091),#5682,.F.);
#93065=ADVANCED_FACE('',(#8092),#5683,.F.);
#93066=ADVANCED_FACE('',(#8093),#5684,.T.);
#93067=ADVANCED_FACE('',(#8094),#5685,.T.);
#93068=ADVANCED_FACE('',(#8095),#6604,.F.);
#93069=ADVANCED_FACE('',(#8096),#136,.F.);
#93070=ADVANCED_FACE('',(#8097),#6605,.F.);
#93071=ADVANCED_FACE('',(#8098),#137,.T.);
#93072=ADVANCED_FACE('',(#8099),#6606,.F.);
#93073=ADVANCED_FACE('',(#8100),#5686,.F.);
#93074=ADVANCED_FACE('',(#8101),#5687,.F.);
#93075=ADVANCED_FACE('',(#8102),#5688,.T.);
#93076=ADVANCED_FACE('',(#8103),#5689,.T.);
#93077=ADVANCED_FACE('',(#8104),#6607,.F.);
#93078=ADVANCED_FACE('',(#8105),#138,.F.);
#93079=ADVANCED_FACE('',(#8106),#6608,.F.);
#93080=ADVANCED_FACE('',(#8107),#139,.T.);
#93081=ADVANCED_FACE('',(#8108),#6609,.F.);
#93082=ADVANCED_FACE('',(#8109),#5690,.F.);
#93083=ADVANCED_FACE('',(#8110),#5691,.F.);
#93084=ADVANCED_FACE('',(#8111),#5692,.T.);
#93085=ADVANCED_FACE('',(#8112),#5693,.T.);
#93086=ADVANCED_FACE('',(#8113),#6610,.F.);
#93087=ADVANCED_FACE('',(#8114),#140,.F.);
#93088=ADVANCED_FACE('',(#8115),#6611,.F.);
#93089=ADVANCED_FACE('',(#8116),#141,.T.);
#93090=ADVANCED_FACE('',(#8117),#6612,.F.);
#93091=ADVANCED_FACE('',(#8118),#5694,.F.);
#93092=ADVANCED_FACE('',(#8119),#5695,.F.);
#93093=ADVANCED_FACE('',(#8120),#5696,.T.);
#93094=ADVANCED_FACE('',(#8121),#5697,.T.);
#93095=ADVANCED_FACE('',(#8122),#6613,.F.);
#93096=ADVANCED_FACE('',(#8123),#142,.F.);
#93097=ADVANCED_FACE('',(#8124),#6614,.F.);
#93098=ADVANCED_FACE('',(#8125),#143,.T.);
#93099=ADVANCED_FACE('',(#8126),#6615,.F.);
#93100=ADVANCED_FACE('',(#8127),#5698,.F.);
#93101=ADVANCED_FACE('',(#8128),#5699,.F.);
#93102=ADVANCED_FACE('',(#8129),#5700,.T.);
#93103=ADVANCED_FACE('',(#8130),#5701,.T.);
#93104=ADVANCED_FACE('',(#8131),#6616,.F.);
#93105=ADVANCED_FACE('',(#8132),#144,.F.);
#93106=ADVANCED_FACE('',(#8133),#6617,.F.);
#93107=ADVANCED_FACE('',(#8134),#145,.T.);
#93108=ADVANCED_FACE('',(#8135),#6618,.F.);
#93109=ADVANCED_FACE('',(#8136),#5702,.F.);
#93110=ADVANCED_FACE('',(#8137),#5703,.F.);
#93111=ADVANCED_FACE('',(#8138),#5704,.T.);
#93112=ADVANCED_FACE('',(#8139),#5705,.T.);
#93113=ADVANCED_FACE('',(#8140),#6619,.F.);
#93114=ADVANCED_FACE('',(#8141),#146,.F.);
#93115=ADVANCED_FACE('',(#8142),#6620,.F.);
#93116=ADVANCED_FACE('',(#8143),#147,.T.);
#93117=ADVANCED_FACE('',(#8144),#6621,.F.);
#93118=ADVANCED_FACE('',(#8145),#5706,.F.);
#93119=ADVANCED_FACE('',(#8146),#5707,.F.);
#93120=ADVANCED_FACE('',(#8147),#5708,.T.);
#93121=ADVANCED_FACE('',(#8148),#5709,.T.);
#93122=ADVANCED_FACE('',(#8149),#6622,.F.);
#93123=ADVANCED_FACE('',(#8150),#148,.F.);
#93124=ADVANCED_FACE('',(#8151),#6623,.F.);
#93125=ADVANCED_FACE('',(#8152),#149,.T.);
#93126=ADVANCED_FACE('',(#8153),#6624,.F.);
#93127=ADVANCED_FACE('',(#8154),#5710,.F.);
#93128=ADVANCED_FACE('',(#8155),#5711,.F.);
#93129=ADVANCED_FACE('',(#8156),#5712,.T.);
#93130=ADVANCED_FACE('',(#8157),#5713,.T.);
#93131=ADVANCED_FACE('',(#8158),#6625,.F.);
#93132=ADVANCED_FACE('',(#8159),#150,.F.);
#93133=ADVANCED_FACE('',(#8160),#6626,.F.);
#93134=ADVANCED_FACE('',(#8161),#151,.T.);
#93135=ADVANCED_FACE('',(#8162),#6627,.F.);
#93136=ADVANCED_FACE('',(#8163),#5714,.F.);
#93137=ADVANCED_FACE('',(#8164),#5715,.F.);
#93138=ADVANCED_FACE('',(#8165),#5716,.T.);
#93139=ADVANCED_FACE('',(#8166),#5717,.T.);
#93140=ADVANCED_FACE('',(#8167),#6628,.F.);
#93141=ADVANCED_FACE('',(#8168),#152,.F.);
#93142=ADVANCED_FACE('',(#8169),#6629,.F.);
#93143=ADVANCED_FACE('',(#8170),#153,.T.);
#93144=ADVANCED_FACE('',(#8171),#6630,.F.);
#93145=ADVANCED_FACE('',(#8172),#5718,.F.);
#93146=ADVANCED_FACE('',(#8173),#5719,.F.);
#93147=ADVANCED_FACE('',(#8174),#5720,.T.);
#93148=ADVANCED_FACE('',(#8175),#5721,.T.);
#93149=ADVANCED_FACE('',(#8176),#6631,.F.);
#93150=ADVANCED_FACE('',(#8177),#154,.F.);
#93151=ADVANCED_FACE('',(#8178),#6632,.F.);
#93152=ADVANCED_FACE('',(#8179),#155,.T.);
#93153=ADVANCED_FACE('',(#8180),#6633,.F.);
#93154=ADVANCED_FACE('',(#8181),#5722,.F.);
#93155=ADVANCED_FACE('',(#8182),#5723,.F.);
#93156=ADVANCED_FACE('',(#8183),#5724,.T.);
#93157=ADVANCED_FACE('',(#8184),#5725,.T.);
#93158=ADVANCED_FACE('',(#8185),#6634,.F.);
#93159=ADVANCED_FACE('',(#8186),#156,.F.);
#93160=ADVANCED_FACE('',(#8187),#6635,.F.);
#93161=ADVANCED_FACE('',(#8188),#157,.T.);
#93162=ADVANCED_FACE('',(#8189),#6636,.F.);
#93163=ADVANCED_FACE('',(#8190),#5726,.F.);
#93164=ADVANCED_FACE('',(#8191),#5727,.F.);
#93165=ADVANCED_FACE('',(#8192),#5728,.T.);
#93166=ADVANCED_FACE('',(#8193),#5729,.T.);
#93167=ADVANCED_FACE('',(#8194),#6637,.F.);
#93168=ADVANCED_FACE('',(#8195),#158,.F.);
#93169=ADVANCED_FACE('',(#8196),#6638,.F.);
#93170=ADVANCED_FACE('',(#8197),#159,.T.);
#93171=ADVANCED_FACE('',(#8198),#6639,.F.);
#93172=ADVANCED_FACE('',(#8199),#5730,.F.);
#93173=ADVANCED_FACE('',(#8200),#5731,.F.);
#93174=ADVANCED_FACE('',(#8201),#5732,.T.);
#93175=ADVANCED_FACE('',(#8202),#5733,.T.);
#93176=ADVANCED_FACE('',(#8203),#6640,.F.);
#93177=ADVANCED_FACE('',(#8204),#160,.F.);
#93178=ADVANCED_FACE('',(#8205),#6641,.F.);
#93179=ADVANCED_FACE('',(#8206),#161,.T.);
#93180=ADVANCED_FACE('',(#8207),#6642,.F.);
#93181=ADVANCED_FACE('',(#8208),#5734,.F.);
#93182=ADVANCED_FACE('',(#8209),#5735,.F.);
#93183=ADVANCED_FACE('',(#8210),#5736,.T.);
#93184=ADVANCED_FACE('',(#8211),#5737,.T.);
#93185=ADVANCED_FACE('',(#8212),#6643,.F.);
#93186=ADVANCED_FACE('',(#8213),#162,.F.);
#93187=ADVANCED_FACE('',(#8214),#6644,.F.);
#93188=ADVANCED_FACE('',(#8215),#163,.T.);
#93189=ADVANCED_FACE('',(#8216),#6645,.F.);
#93190=ADVANCED_FACE('',(#8217),#5738,.F.);
#93191=ADVANCED_FACE('',(#8218),#5739,.F.);
#93192=ADVANCED_FACE('',(#8219),#5740,.T.);
#93193=ADVANCED_FACE('',(#8220),#5741,.T.);
#93194=ADVANCED_FACE('',(#8221),#6646,.F.);
#93195=ADVANCED_FACE('',(#8222),#164,.F.);
#93196=ADVANCED_FACE('',(#8223),#6647,.F.);
#93197=ADVANCED_FACE('',(#8224),#165,.T.);
#93198=ADVANCED_FACE('',(#8225),#6648,.F.);
#93199=ADVANCED_FACE('',(#8226),#5742,.F.);
#93200=ADVANCED_FACE('',(#8227),#5743,.F.);
#93201=ADVANCED_FACE('',(#8228),#5744,.T.);
#93202=ADVANCED_FACE('',(#8229),#5745,.T.);
#93203=ADVANCED_FACE('',(#8230),#6649,.F.);
#93204=ADVANCED_FACE('',(#8231),#166,.F.);
#93205=ADVANCED_FACE('',(#8232),#6650,.F.);
#93206=ADVANCED_FACE('',(#8233),#167,.T.);
#93207=ADVANCED_FACE('',(#8234),#6651,.F.);
#93208=ADVANCED_FACE('',(#8235),#5746,.F.);
#93209=ADVANCED_FACE('',(#8236),#5747,.F.);
#93210=ADVANCED_FACE('',(#8237),#5748,.T.);
#93211=ADVANCED_FACE('',(#8238),#5749,.T.);
#93212=ADVANCED_FACE('',(#8239),#6652,.F.);
#93213=ADVANCED_FACE('',(#8240),#168,.F.);
#93214=ADVANCED_FACE('',(#8241),#6653,.F.);
#93215=ADVANCED_FACE('',(#8242),#169,.T.);
#93216=ADVANCED_FACE('',(#8243),#6654,.F.);
#93217=ADVANCED_FACE('',(#8244),#5750,.F.);
#93218=ADVANCED_FACE('',(#8245),#5751,.F.);
#93219=ADVANCED_FACE('',(#8246),#5752,.T.);
#93220=ADVANCED_FACE('',(#8247),#5753,.T.);
#93221=ADVANCED_FACE('',(#8248),#6655,.F.);
#93222=ADVANCED_FACE('',(#8249),#170,.F.);
#93223=ADVANCED_FACE('',(#8250),#6656,.F.);
#93224=ADVANCED_FACE('',(#8251),#171,.T.);
#93225=ADVANCED_FACE('',(#8252),#6657,.F.);
#93226=ADVANCED_FACE('',(#8253),#5754,.F.);
#93227=ADVANCED_FACE('',(#8254),#5755,.F.);
#93228=ADVANCED_FACE('',(#8255),#5756,.T.);
#93229=ADVANCED_FACE('',(#8256),#5757,.T.);
#93230=ADVANCED_FACE('',(#8257),#6658,.F.);
#93231=ADVANCED_FACE('',(#8258),#172,.F.);
#93232=ADVANCED_FACE('',(#8259),#6659,.F.);
#93233=ADVANCED_FACE('',(#8260),#173,.T.);
#93234=ADVANCED_FACE('',(#8261),#6660,.F.);
#93235=ADVANCED_FACE('',(#8262),#5758,.F.);
#93236=ADVANCED_FACE('',(#8263),#5759,.F.);
#93237=ADVANCED_FACE('',(#8264),#5760,.T.);
#93238=ADVANCED_FACE('',(#8265),#5761,.T.);
#93239=ADVANCED_FACE('',(#8266),#6661,.F.);
#93240=ADVANCED_FACE('',(#8267),#174,.F.);
#93241=ADVANCED_FACE('',(#8268),#6662,.F.);
#93242=ADVANCED_FACE('',(#8269),#175,.T.);
#93243=ADVANCED_FACE('',(#8270),#6663,.F.);
#93244=ADVANCED_FACE('',(#8271),#5762,.F.);
#93245=ADVANCED_FACE('',(#8272),#5763,.F.);
#93246=ADVANCED_FACE('',(#8273),#5764,.T.);
#93247=ADVANCED_FACE('',(#8274),#5765,.T.);
#93248=ADVANCED_FACE('',(#8275),#6664,.F.);
#93249=ADVANCED_FACE('',(#8276),#176,.F.);
#93250=ADVANCED_FACE('',(#8277),#6665,.F.);
#93251=ADVANCED_FACE('',(#8278),#177,.T.);
#93252=ADVANCED_FACE('',(#8279),#6666,.F.);
#93253=ADVANCED_FACE('',(#8280),#5766,.F.);
#93254=ADVANCED_FACE('',(#8281),#5767,.F.);
#93255=ADVANCED_FACE('',(#8282),#5768,.T.);
#93256=ADVANCED_FACE('',(#8283),#5769,.T.);
#93257=ADVANCED_FACE('',(#8284),#6667,.F.);
#93258=ADVANCED_FACE('',(#8285),#178,.F.);
#93259=ADVANCED_FACE('',(#8286),#6668,.F.);
#93260=ADVANCED_FACE('',(#8287),#179,.T.);
#93261=ADVANCED_FACE('',(#8288),#6669,.F.);
#93262=ADVANCED_FACE('',(#8289),#5770,.F.);
#93263=ADVANCED_FACE('',(#8290),#5771,.F.);
#93264=ADVANCED_FACE('',(#8291),#5772,.T.);
#93265=ADVANCED_FACE('',(#8292),#5773,.T.);
#93266=ADVANCED_FACE('',(#8293),#6670,.F.);
#93267=ADVANCED_FACE('',(#8294),#180,.F.);
#93268=ADVANCED_FACE('',(#8295),#6671,.F.);
#93269=ADVANCED_FACE('',(#8296),#181,.T.);
#93270=ADVANCED_FACE('',(#8297),#6672,.F.);
#93271=ADVANCED_FACE('',(#8298),#5774,.F.);
#93272=ADVANCED_FACE('',(#8299),#5775,.F.);
#93273=ADVANCED_FACE('',(#8300),#5776,.T.);
#93274=ADVANCED_FACE('',(#8301),#5777,.T.);
#93275=ADVANCED_FACE('',(#8302),#6673,.F.);
#93276=ADVANCED_FACE('',(#8303),#182,.F.);
#93277=ADVANCED_FACE('',(#8304),#6674,.F.);
#93278=ADVANCED_FACE('',(#8305),#183,.T.);
#93279=ADVANCED_FACE('',(#8306),#6675,.F.);
#93280=ADVANCED_FACE('',(#8307),#5778,.F.);
#93281=ADVANCED_FACE('',(#8308),#5779,.F.);
#93282=ADVANCED_FACE('',(#8309),#5780,.T.);
#93283=ADVANCED_FACE('',(#8310),#5781,.T.);
#93284=ADVANCED_FACE('',(#8311),#6676,.F.);
#93285=ADVANCED_FACE('',(#8312),#184,.F.);
#93286=ADVANCED_FACE('',(#8313),#6677,.F.);
#93287=ADVANCED_FACE('',(#8314),#185,.T.);
#93288=ADVANCED_FACE('',(#8315),#6678,.F.);
#93289=ADVANCED_FACE('',(#8316),#5782,.F.);
#93290=ADVANCED_FACE('',(#8317),#5783,.F.);
#93291=ADVANCED_FACE('',(#8318),#5784,.T.);
#93292=ADVANCED_FACE('',(#8319),#5785,.T.);
#93293=ADVANCED_FACE('',(#8320,#6366),#6679,.F.);
#93294=ADVANCED_FACE('',(#8321),#6680,.F.);
#93295=ADVANCED_FACE('',(#8322),#186,.F.);
#93296=ADVANCED_FACE('',(#8323),#6681,.F.);
#93297=ADVANCED_FACE('',(#8324),#187,.T.);
#93298=ADVANCED_FACE('',(#8325),#6682,.F.);
#93299=ADVANCED_FACE('',(#8326,#6367),#6683,.F.);
#93300=ADVANCED_FACE('',(#8327,#6368),#6684,.F.);
#93301=ADVANCED_FACE('',(#8328),#5786,.F.);
#93302=ADVANCED_FACE('',(#8329),#5787,.F.);
#93303=ADVANCED_FACE('',(#8330),#5788,.T.);
#93304=ADVANCED_FACE('',(#8331),#5789,.T.);
#93305=ADVANCED_FACE('',(#8332),#6685,.F.);
#93306=ADVANCED_FACE('',(#8333),#6686,.T.);
#93307=ADVANCED_FACE('',(#8334),#6687,.F.);
#93308=ADVANCED_FACE('',(#8335),#90367,.T.);
#93309=ADVANCED_FACE('',(#8336),#90368,.T.);
#93310=ADVANCED_FACE('',(#8337),#90369,.F.);
#93311=ADVANCED_FACE('',(#8338),#2506,.F.);
#93312=ADVANCED_FACE('',(#8339),#90370,.F.);
#93313=ADVANCED_FACE('',(#8340),#90371,.F.);
#93314=ADVANCED_FACE('',(#8341),#2507,.F.);
#93315=ADVANCED_FACE('',(#8342),#2508,.F.);
#93316=ADVANCED_FACE('',(#8343),#90372,.F.);
#93317=ADVANCED_FACE('',(#8344),#90373,.F.);
#93318=ADVANCED_FACE('',(#8345),#2509,.F.);
#93319=ADVANCED_FACE('',(#8346),#90374,.F.);
#93320=ADVANCED_FACE('',(#8347),#5790,.F.);
#93321=ADVANCED_FACE('',(#8348),#2510,.F.);
#93322=ADVANCED_FACE('',(#8349),#2511,.F.);
#93323=ADVANCED_FACE('',(#8350),#90375,.F.);
#93324=ADVANCED_FACE('',(#8351),#90376,.F.);
#93325=ADVANCED_FACE('',(#8352),#2512,.F.);
#93326=ADVANCED_FACE('',(#8353),#2513,.F.);
#93327=ADVANCED_FACE('',(#8354),#5791,.F.);
#93328=ADVANCED_FACE('',(#8355),#90377,.F.);
#93329=ADVANCED_FACE('',(#8356),#2514,.F.);
#93330=ADVANCED_FACE('',(#8357),#90378,.F.);
#93331=ADVANCED_FACE('',(#8358),#90379,.F.);
#93332=ADVANCED_FACE('',(#8359),#2515,.F.);
#93333=ADVANCED_FACE('',(#8360),#2516,.F.);
#93334=ADVANCED_FACE('',(#8361),#90380,.F.);
#93335=ADVANCED_FACE('',(#8362),#90381,.F.);
#93336=ADVANCED_FACE('',(#8363),#2517,.F.);
#93337=ADVANCED_FACE('',(#8364),#90382,.F.);
#93338=ADVANCED_FACE('',(#8365),#6688,.F.);
#93339=ADVANCED_FACE('',(#8366),#6689,.T.);
#93340=ADVANCED_FACE('',(#8367),#6690,.F.);
#93341=ADVANCED_FACE('',(#8368),#6691,.F.);
#93342=ADVANCED_FACE('',(#8369),#6692,.T.);
#93343=ADVANCED_FACE('',(#8370),#6693,.F.);
#93344=ADVANCED_FACE('',(#8371),#6694,.F.);
#93345=ADVANCED_FACE('',(#8372),#6695,.T.);
#93346=ADVANCED_FACE('',(#8373),#6696,.F.);
#93347=ADVANCED_FACE('',(#8374),#6697,.F.);
#93348=ADVANCED_FACE('',(#8375),#6698,.T.);
#93349=ADVANCED_FACE('',(#8376),#6699,.F.);
#93350=ADVANCED_FACE('',(#8377),#6700,.F.);
#93351=ADVANCED_FACE('',(#8378),#6701,.T.);
#93352=ADVANCED_FACE('',(#8379),#6702,.F.);
#93353=ADVANCED_FACE('',(#8380),#6703,.F.);
#93354=ADVANCED_FACE('',(#8381),#6704,.T.);
#93355=ADVANCED_FACE('',(#8382),#6705,.F.);
#93356=ADVANCED_FACE('',(#8383),#6706,.F.);
#93357=ADVANCED_FACE('',(#8384),#6707,.T.);
#93358=ADVANCED_FACE('',(#8385),#6708,.F.);
#93359=ADVANCED_FACE('',(#8386),#6709,.F.);
#93360=ADVANCED_FACE('',(#8387),#6710,.T.);
#93361=ADVANCED_FACE('',(#8388),#6711,.F.);
#93362=ADVANCED_FACE('',(#8389),#6712,.F.);
#93363=ADVANCED_FACE('',(#8390),#6713,.T.);
#93364=ADVANCED_FACE('',(#8391),#6714,.F.);
#93365=ADVANCED_FACE('',(#8392),#6715,.F.);
#93366=ADVANCED_FACE('',(#8393),#6716,.T.);
#93367=ADVANCED_FACE('',(#8394),#6717,.F.);
#93368=ADVANCED_FACE('',(#8395),#6718,.F.);
#93369=ADVANCED_FACE('',(#8396),#6719,.T.);
#93370=ADVANCED_FACE('',(#8397),#6720,.F.);
#93371=ADVANCED_FACE('',(#8398),#6721,.F.);
#93372=ADVANCED_FACE('',(#8399),#6722,.T.);
#93373=ADVANCED_FACE('',(#8400),#6723,.F.);
#93374=ADVANCED_FACE('',(#8401),#6724,.F.);
#93375=ADVANCED_FACE('',(#8402),#6725,.T.);
#93376=ADVANCED_FACE('',(#8403),#6726,.F.);
#93377=ADVANCED_FACE('',(#8404),#6727,.F.);
#93378=ADVANCED_FACE('',(#8405),#6728,.T.);
#93379=ADVANCED_FACE('',(#8406),#6729,.F.);
#93380=ADVANCED_FACE('',(#8407),#6730,.F.);
#93381=ADVANCED_FACE('',(#8408),#6731,.T.);
#93382=ADVANCED_FACE('',(#8409),#6732,.F.);
#93383=ADVANCED_FACE('',(#8410),#6733,.F.);
#93384=ADVANCED_FACE('',(#8411),#6734,.T.);
#93385=ADVANCED_FACE('',(#8412),#6735,.F.);
#93386=ADVANCED_FACE('',(#8413),#6736,.F.);
#93387=ADVANCED_FACE('',(#8414),#6737,.T.);
#93388=ADVANCED_FACE('',(#8415),#6738,.F.);
#93389=ADVANCED_FACE('',(#8416),#6739,.F.);
#93390=ADVANCED_FACE('',(#8417),#6740,.T.);
#93391=ADVANCED_FACE('',(#8418),#6741,.F.);
#93392=ADVANCED_FACE('',(#8419),#6742,.F.);
#93393=ADVANCED_FACE('',(#8420),#6743,.T.);
#93394=ADVANCED_FACE('',(#8421),#6744,.F.);
#93395=ADVANCED_FACE('',(#8422),#6745,.F.);
#93396=ADVANCED_FACE('',(#8423),#6746,.T.);
#93397=ADVANCED_FACE('',(#8424),#6747,.F.);
#93398=ADVANCED_FACE('',(#8425),#6748,.F.);
#93399=ADVANCED_FACE('',(#8426),#6749,.T.);
#93400=ADVANCED_FACE('',(#8427),#6750,.F.);
#93401=ADVANCED_FACE('',(#8428),#6751,.F.);
#93402=ADVANCED_FACE('',(#8429),#6752,.T.);
#93403=ADVANCED_FACE('',(#8430),#6753,.F.);
#93404=ADVANCED_FACE('',(#8431),#6754,.F.);
#93405=ADVANCED_FACE('',(#8432),#6755,.T.);
#93406=ADVANCED_FACE('',(#8433),#6756,.F.);
#93407=ADVANCED_FACE('',(#8434),#6757,.F.);
#93408=ADVANCED_FACE('',(#8435),#6758,.T.);
#93409=ADVANCED_FACE('',(#8436),#6759,.F.);
#93410=ADVANCED_FACE('',(#8437),#6760,.F.);
#93411=ADVANCED_FACE('',(#8438),#6761,.T.);
#93412=ADVANCED_FACE('',(#8439),#6762,.F.);
#93413=ADVANCED_FACE('',(#8440),#6763,.F.);
#93414=ADVANCED_FACE('',(#8441),#6764,.T.);
#93415=ADVANCED_FACE('',(#8442),#6765,.F.);
#93416=ADVANCED_FACE('',(#8443),#6766,.F.);
#93417=ADVANCED_FACE('',(#8444),#6767,.T.);
#93418=ADVANCED_FACE('',(#8445),#6768,.F.);
#93419=ADVANCED_FACE('',(#8446),#6769,.F.);
#93420=ADVANCED_FACE('',(#8447),#6770,.T.);
#93421=ADVANCED_FACE('',(#8448),#6771,.F.);
#93422=ADVANCED_FACE('',(#8449),#6772,.F.);
#93423=ADVANCED_FACE('',(#8450),#6773,.T.);
#93424=ADVANCED_FACE('',(#8451),#6774,.F.);
#93425=ADVANCED_FACE('',(#8452),#6775,.F.);
#93426=ADVANCED_FACE('',(#8453),#6776,.T.);
#93427=ADVANCED_FACE('',(#8454),#6777,.F.);
#93428=ADVANCED_FACE('',(#8455),#6778,.F.);
#93429=ADVANCED_FACE('',(#8456),#6779,.T.);
#93430=ADVANCED_FACE('',(#8457),#6780,.F.);
#93431=ADVANCED_FACE('',(#8458),#6781,.F.);
#93432=ADVANCED_FACE('',(#8459),#6782,.T.);
#93433=ADVANCED_FACE('',(#8460),#6783,.F.);
#93434=ADVANCED_FACE('',(#8461),#6784,.F.);
#93435=ADVANCED_FACE('',(#8462),#6785,.T.);
#93436=ADVANCED_FACE('',(#8463),#6786,.F.);
#93437=ADVANCED_FACE('',(#8464),#6787,.F.);
#93438=ADVANCED_FACE('',(#8465),#6788,.T.);
#93439=ADVANCED_FACE('',(#8466),#6789,.F.);
#93440=ADVANCED_FACE('',(#8467),#6790,.F.);
#93441=ADVANCED_FACE('',(#8468),#6791,.T.);
#93442=ADVANCED_FACE('',(#8469),#6792,.F.);
#93443=ADVANCED_FACE('',(#8470),#6793,.F.);
#93444=ADVANCED_FACE('',(#8471),#6794,.T.);
#93445=ADVANCED_FACE('',(#8472),#6795,.F.);
#93446=ADVANCED_FACE('',(#8473),#6796,.F.);
#93447=ADVANCED_FACE('',(#8474),#6797,.T.);
#93448=ADVANCED_FACE('',(#8475),#6798,.F.);
#93449=ADVANCED_FACE('',(#8476),#6799,.F.);
#93450=ADVANCED_FACE('',(#8477),#6800,.T.);
#93451=ADVANCED_FACE('',(#8478),#6801,.F.);
#93452=ADVANCED_FACE('',(#8479),#6802,.F.);
#93453=ADVANCED_FACE('',(#8480),#6803,.T.);
#93454=ADVANCED_FACE('',(#8481),#6804,.F.);
#93455=ADVANCED_FACE('',(#8482),#6805,.F.);
#93456=ADVANCED_FACE('',(#8483),#6806,.T.);
#93457=ADVANCED_FACE('',(#8484),#6807,.F.);
#93458=ADVANCED_FACE('',(#8485),#6808,.F.);
#93459=ADVANCED_FACE('',(#8486),#6809,.T.);
#93460=ADVANCED_FACE('',(#8487),#6810,.F.);
#93461=ADVANCED_FACE('',(#8488),#6811,.F.);
#93462=ADVANCED_FACE('',(#8489),#6812,.T.);
#93463=ADVANCED_FACE('',(#8490),#6813,.F.);
#93464=ADVANCED_FACE('',(#8491),#6814,.F.);
#93465=ADVANCED_FACE('',(#8492),#6815,.T.);
#93466=ADVANCED_FACE('',(#8493),#6816,.F.);
#93467=ADVANCED_FACE('',(#8494),#6817,.F.);
#93468=ADVANCED_FACE('',(#8495),#6818,.T.);
#93469=ADVANCED_FACE('',(#8496),#6819,.F.);
#93470=ADVANCED_FACE('',(#8497),#6820,.F.);
#93471=ADVANCED_FACE('',(#8498),#6821,.T.);
#93472=ADVANCED_FACE('',(#8499),#6822,.F.);
#93473=ADVANCED_FACE('',(#8500),#6823,.F.);
#93474=ADVANCED_FACE('',(#8501),#6824,.T.);
#93475=ADVANCED_FACE('',(#8502),#6825,.F.);
#93476=ADVANCED_FACE('',(#8503),#6826,.F.);
#93477=ADVANCED_FACE('',(#8504),#6827,.T.);
#93478=ADVANCED_FACE('',(#8505),#6828,.F.);
#93479=ADVANCED_FACE('',(#8506),#6829,.F.);
#93480=ADVANCED_FACE('',(#8507),#6830,.T.);
#93481=ADVANCED_FACE('',(#8508),#6831,.F.);
#93482=ADVANCED_FACE('',(#8509),#6832,.F.);
#93483=ADVANCED_FACE('',(#8510),#6833,.T.);
#93484=ADVANCED_FACE('',(#8511),#6834,.F.);
#93485=ADVANCED_FACE('',(#8512),#6835,.F.);
#93486=ADVANCED_FACE('',(#8513),#6836,.T.);
#93487=ADVANCED_FACE('',(#8514),#6837,.F.);
#93488=ADVANCED_FACE('',(#8515),#6838,.F.);
#93489=ADVANCED_FACE('',(#8516),#6839,.T.);
#93490=ADVANCED_FACE('',(#8517),#6840,.F.);
#93491=ADVANCED_FACE('',(#8518),#6841,.F.);
#93492=ADVANCED_FACE('',(#8519),#6842,.T.);
#93493=ADVANCED_FACE('',(#8520),#6843,.F.);
#93494=ADVANCED_FACE('',(#8521),#6844,.F.);
#93495=ADVANCED_FACE('',(#8522),#6845,.T.);
#93496=ADVANCED_FACE('',(#8523),#6846,.F.);
#93497=ADVANCED_FACE('',(#8524),#6847,.F.);
#93498=ADVANCED_FACE('',(#8525),#6848,.T.);
#93499=ADVANCED_FACE('',(#8526),#6849,.F.);
#93500=ADVANCED_FACE('',(#8527),#6850,.F.);
#93501=ADVANCED_FACE('',(#8528),#6851,.T.);
#93502=ADVANCED_FACE('',(#8529),#6852,.F.);
#93503=ADVANCED_FACE('',(#8530),#6853,.F.);
#93504=ADVANCED_FACE('',(#8531),#6854,.T.);
#93505=ADVANCED_FACE('',(#8532),#6855,.F.);
#93506=ADVANCED_FACE('',(#8533),#6856,.F.);
#93507=ADVANCED_FACE('',(#8534),#6857,.T.);
#93508=ADVANCED_FACE('',(#8535),#6858,.F.);
#93509=ADVANCED_FACE('',(#8536),#6859,.F.);
#93510=ADVANCED_FACE('',(#8537),#6860,.T.);
#93511=ADVANCED_FACE('',(#8538),#6861,.F.);
#93512=ADVANCED_FACE('',(#8539),#6862,.F.);
#93513=ADVANCED_FACE('',(#8540),#6863,.T.);
#93514=ADVANCED_FACE('',(#8541),#6864,.F.);
#93515=ADVANCED_FACE('',(#8542),#90383,.T.);
#93516=ADVANCED_FACE('',(#8543),#90384,.T.);
#93517=ADVANCED_FACE('',(#8544),#90385,.T.);
#93518=ADVANCED_FACE('',(#8545),#90386,.T.);
#93519=ADVANCED_FACE('',(#8546),#90387,.T.);
#93520=ADVANCED_FACE('',(#8547),#90388,.T.);
#93521=ADVANCED_FACE('',(#8548),#90389,.T.);
#93522=ADVANCED_FACE('',(#8549),#90390,.T.);
#93523=ADVANCED_FACE('',(#8550),#90391,.T.);
#93524=ADVANCED_FACE('',(#8551),#90392,.T.);
#93525=ADVANCED_FACE('',(#8552),#90393,.T.);
#93526=ADVANCED_FACE('',(#8553),#90394,.T.);
#93527=ADVANCED_FACE('',(#8554),#90395,.T.);
#93528=ADVANCED_FACE('',(#8555),#90396,.T.);
#93529=ADVANCED_FACE('',(#8556),#90397,.T.);
#93530=ADVANCED_FACE('',(#8557),#90398,.T.);
#93531=ADVANCED_FACE('',(#8558),#90399,.T.);
#93532=ADVANCED_FACE('',(#8559),#90400,.T.);
#93533=ADVANCED_FACE('',(#8560),#90401,.T.);
#93534=ADVANCED_FACE('',(#8561),#90402,.T.);
#93535=ADVANCED_FACE('',(#8562),#90403,.T.);
#93536=ADVANCED_FACE('',(#8563),#90404,.T.);
#93537=ADVANCED_FACE('',(#8564),#90405,.T.);
#93538=ADVANCED_FACE('',(#8565),#90406,.T.);
#93539=ADVANCED_FACE('',(#8566),#90407,.T.);
#93540=ADVANCED_FACE('',(#8567),#90408,.T.);
#93541=ADVANCED_FACE('',(#8568),#90409,.T.);
#93542=ADVANCED_FACE('',(#8569),#90410,.T.);
#93543=ADVANCED_FACE('',(#8570),#90411,.T.);
#93544=ADVANCED_FACE('',(#8571),#90412,.T.);
#93545=ADVANCED_FACE('',(#8572),#90413,.T.);
#93546=ADVANCED_FACE('',(#8573),#90414,.T.);
#93547=ADVANCED_FACE('',(#8574),#90415,.T.);
#93548=ADVANCED_FACE('',(#8575),#90416,.T.);
#93549=ADVANCED_FACE('',(#8576),#90417,.T.);
#93550=ADVANCED_FACE('',(#8577),#90418,.T.);
#93551=ADVANCED_FACE('',(#8578),#90419,.T.);
#93552=ADVANCED_FACE('',(#8579),#90420,.T.);
#93553=ADVANCED_FACE('',(#8580),#90421,.T.);
#93554=ADVANCED_FACE('',(#8581),#90422,.T.);
#93555=ADVANCED_FACE('',(#8582),#90423,.T.);
#93556=ADVANCED_FACE('',(#8583),#90424,.T.);
#93557=ADVANCED_FACE('',(#8584),#90425,.T.);
#93558=ADVANCED_FACE('',(#8585),#90426,.T.);
#93559=ADVANCED_FACE('',(#8586),#90427,.T.);
#93560=ADVANCED_FACE('',(#8587),#90428,.T.);
#93561=ADVANCED_FACE('',(#8588),#90429,.T.);
#93562=ADVANCED_FACE('',(#8589),#90430,.T.);
#93563=ADVANCED_FACE('',(#8590),#90431,.T.);
#93564=ADVANCED_FACE('',(#8591),#90432,.T.);
#93565=ADVANCED_FACE('',(#8592),#90433,.T.);
#93566=ADVANCED_FACE('',(#8593),#90434,.T.);
#93567=ADVANCED_FACE('',(#8594),#90435,.T.);
#93568=ADVANCED_FACE('',(#8595),#90436,.T.);
#93569=ADVANCED_FACE('',(#8596),#90437,.T.);
#93570=ADVANCED_FACE('',(#8597),#90438,.T.);
#93571=ADVANCED_FACE('',(#8598),#90439,.T.);
#93572=ADVANCED_FACE('',(#8599),#90440,.T.);
#93573=ADVANCED_FACE('',(#8600),#90441,.T.);
#93574=ADVANCED_FACE('',(#8601),#90442,.T.);
#93575=ADVANCED_FACE('',(#8602),#90443,.T.);
#93576=ADVANCED_FACE('',(#8603),#90444,.T.);
#93577=ADVANCED_FACE('',(#8604),#90445,.T.);
#93578=ADVANCED_FACE('',(#8605),#90446,.T.);
#93579=ADVANCED_FACE('',(#8606),#90447,.T.);
#93580=ADVANCED_FACE('',(#8607),#90448,.T.);
#93581=ADVANCED_FACE('',(#8608),#90449,.T.);
#93582=ADVANCED_FACE('',(#8609),#90450,.T.);
#93583=ADVANCED_FACE('',(#8610),#90451,.T.);
#93584=ADVANCED_FACE('',(#8611),#90452,.T.);
#93585=ADVANCED_FACE('',(#8612),#90453,.T.);
#93586=ADVANCED_FACE('',(#8613),#90454,.T.);
#93587=ADVANCED_FACE('',(#8614),#90455,.T.);
#93588=ADVANCED_FACE('',(#8615),#90456,.T.);
#93589=ADVANCED_FACE('',(#8616),#90457,.T.);
#93590=ADVANCED_FACE('',(#8617),#90458,.T.);
#93591=ADVANCED_FACE('',(#8618),#90459,.T.);
#93592=ADVANCED_FACE('',(#8619),#90460,.T.);
#93593=ADVANCED_FACE('',(#8620),#90461,.T.);
#93594=ADVANCED_FACE('',(#8621),#90462,.T.);
#93595=ADVANCED_FACE('',(#8622),#90463,.T.);
#93596=ADVANCED_FACE('',(#8623),#90464,.T.);
#93597=ADVANCED_FACE('',(#8624),#90465,.T.);
#93598=ADVANCED_FACE('',(#8625),#90466,.T.);
#93599=ADVANCED_FACE('',(#8626),#90467,.T.);
#93600=ADVANCED_FACE('',(#8627),#90468,.T.);
#93601=ADVANCED_FACE('',(#8628),#90469,.T.);
#93602=ADVANCED_FACE('',(#8629),#90470,.T.);
#93603=ADVANCED_FACE('',(#8630),#90471,.T.);
#93604=ADVANCED_FACE('',(#8631),#90472,.T.);
#93605=ADVANCED_FACE('',(#8632),#90473,.T.);
#93606=ADVANCED_FACE('',(#8633),#90474,.T.);
#93607=ADVANCED_FACE('',(#8634),#90475,.T.);
#93608=ADVANCED_FACE('',(#8635),#90476,.T.);
#93609=ADVANCED_FACE('',(#8636),#90477,.T.);
#93610=ADVANCED_FACE('',(#8637),#90478,.T.);
#93611=ADVANCED_FACE('',(#8638),#90479,.T.);
#93612=ADVANCED_FACE('',(#8639),#90480,.T.);
#93613=ADVANCED_FACE('',(#8640),#90481,.T.);
#93614=ADVANCED_FACE('',(#8641),#90482,.T.);
#93615=ADVANCED_FACE('',(#8642),#90483,.T.);
#93616=ADVANCED_FACE('',(#8643),#90484,.T.);
#93617=ADVANCED_FACE('',(#8644),#90485,.T.);
#93618=ADVANCED_FACE('',(#8645),#90486,.T.);
#93619=ADVANCED_FACE('',(#8646),#90487,.T.);
#93620=ADVANCED_FACE('',(#8647),#90488,.T.);
#93621=ADVANCED_FACE('',(#8648),#90489,.T.);
#93622=ADVANCED_FACE('',(#8649),#90490,.T.);
#93623=ADVANCED_FACE('',(#8650),#90491,.T.);
#93624=ADVANCED_FACE('',(#8651),#90492,.T.);
#93625=ADVANCED_FACE('',(#8652),#90493,.T.);
#93626=ADVANCED_FACE('',(#8653),#90494,.T.);
#93627=ADVANCED_FACE('',(#8654),#90495,.T.);
#93628=ADVANCED_FACE('',(#8655),#90496,.T.);
#93629=ADVANCED_FACE('',(#8656),#90497,.T.);
#93630=ADVANCED_FACE('',(#8657),#90498,.T.);
#93631=ADVANCED_FACE('',(#8658),#90499,.T.);
#93632=ADVANCED_FACE('',(#8659),#90500,.T.);
#93633=ADVANCED_FACE('',(#8660),#90501,.F.);
#93634=ADVANCED_FACE('',(#8661),#2518,.F.);
#93635=ADVANCED_FACE('',(#8662),#90502,.F.);
#93636=ADVANCED_FACE('',(#8663),#90503,.F.);
#93637=ADVANCED_FACE('',(#8664),#2519,.F.);
#93638=ADVANCED_FACE('',(#8665),#2520,.F.);
#93639=ADVANCED_FACE('',(#8666),#90504,.F.);
#93640=ADVANCED_FACE('',(#8667),#90505,.F.);
#93641=ADVANCED_FACE('',(#8668),#2521,.F.);
#93642=ADVANCED_FACE('',(#8669),#90506,.F.);
#93643=ADVANCED_FACE('',(#8670),#5792,.F.);
#93644=ADVANCED_FACE('',(#8671),#2522,.F.);
#93645=ADVANCED_FACE('',(#8672),#2523,.F.);
#93646=ADVANCED_FACE('',(#8673),#90507,.F.);
#93647=ADVANCED_FACE('',(#8674),#90508,.F.);
#93648=ADVANCED_FACE('',(#8675),#2524,.F.);
#93649=ADVANCED_FACE('',(#8676),#2525,.F.);
#93650=ADVANCED_FACE('',(#8677),#5793,.F.);
#93651=ADVANCED_FACE('',(#8678),#90509,.F.);
#93652=ADVANCED_FACE('',(#8679),#2526,.F.);
#93653=ADVANCED_FACE('',(#8680),#90510,.F.);
#93654=ADVANCED_FACE('',(#8681),#90511,.F.);
#93655=ADVANCED_FACE('',(#8682),#2527,.F.);
#93656=ADVANCED_FACE('',(#8683),#2528,.F.);
#93657=ADVANCED_FACE('',(#8684),#90512,.F.);
#93658=ADVANCED_FACE('',(#8685),#90513,.F.);
#93659=ADVANCED_FACE('',(#8686),#2529,.F.);
#93660=ADVANCED_FACE('',(#8687),#90514,.F.);
#93661=ADVANCED_FACE('',(#8688),#90515,.F.);
#93662=ADVANCED_FACE('',(#8689),#2530,.F.);
#93663=ADVANCED_FACE('',(#8690),#90516,.F.);
#93664=ADVANCED_FACE('',(#8691),#90517,.F.);
#93665=ADVANCED_FACE('',(#8692),#2531,.F.);
#93666=ADVANCED_FACE('',(#8693),#2532,.F.);
#93667=ADVANCED_FACE('',(#8694),#90518,.F.);
#93668=ADVANCED_FACE('',(#8695),#90519,.F.);
#93669=ADVANCED_FACE('',(#8696),#2533,.F.);
#93670=ADVANCED_FACE('',(#8697),#90520,.F.);
#93671=ADVANCED_FACE('',(#8698),#5794,.F.);
#93672=ADVANCED_FACE('',(#8699),#2534,.F.);
#93673=ADVANCED_FACE('',(#8700),#2535,.F.);
#93674=ADVANCED_FACE('',(#8701),#90521,.F.);
#93675=ADVANCED_FACE('',(#8702),#90522,.F.);
#93676=ADVANCED_FACE('',(#8703),#2536,.F.);
#93677=ADVANCED_FACE('',(#8704),#2537,.F.);
#93678=ADVANCED_FACE('',(#8705),#5795,.F.);
#93679=ADVANCED_FACE('',(#8706),#90523,.F.);
#93680=ADVANCED_FACE('',(#8707),#2538,.F.);
#93681=ADVANCED_FACE('',(#8708),#90524,.F.);
#93682=ADVANCED_FACE('',(#8709),#90525,.F.);
#93683=ADVANCED_FACE('',(#8710),#2539,.F.);
#93684=ADVANCED_FACE('',(#8711),#2540,.F.);
#93685=ADVANCED_FACE('',(#8712),#90526,.F.);
#93686=ADVANCED_FACE('',(#8713),#90527,.F.);
#93687=ADVANCED_FACE('',(#8714),#2541,.F.);
#93688=ADVANCED_FACE('',(#8715),#90528,.F.);
#93689=ADVANCED_FACE('',(#8716),#90529,.F.);
#93690=ADVANCED_FACE('',(#8717),#2542,.F.);
#93691=ADVANCED_FACE('',(#8718),#90530,.F.);
#93692=ADVANCED_FACE('',(#8719),#90531,.F.);
#93693=ADVANCED_FACE('',(#8720),#2543,.F.);
#93694=ADVANCED_FACE('',(#8721),#2544,.F.);
#93695=ADVANCED_FACE('',(#8722),#90532,.F.);
#93696=ADVANCED_FACE('',(#8723),#90533,.F.);
#93697=ADVANCED_FACE('',(#8724),#2545,.F.);
#93698=ADVANCED_FACE('',(#8725),#90534,.F.);
#93699=ADVANCED_FACE('',(#8726),#5796,.F.);
#93700=ADVANCED_FACE('',(#8727),#2546,.F.);
#93701=ADVANCED_FACE('',(#8728),#2547,.F.);
#93702=ADVANCED_FACE('',(#8729),#90535,.F.);
#93703=ADVANCED_FACE('',(#8730),#90536,.F.);
#93704=ADVANCED_FACE('',(#8731),#2548,.F.);
#93705=ADVANCED_FACE('',(#8732),#2549,.F.);
#93706=ADVANCED_FACE('',(#8733),#5797,.F.);
#93707=ADVANCED_FACE('',(#8734),#90537,.F.);
#93708=ADVANCED_FACE('',(#8735),#2550,.F.);
#93709=ADVANCED_FACE('',(#8736),#90538,.F.);
#93710=ADVANCED_FACE('',(#8737),#90539,.F.);
#93711=ADVANCED_FACE('',(#8738),#2551,.F.);
#93712=ADVANCED_FACE('',(#8739),#2552,.F.);
#93713=ADVANCED_FACE('',(#8740),#90540,.F.);
#93714=ADVANCED_FACE('',(#8741),#90541,.F.);
#93715=ADVANCED_FACE('',(#8742),#2553,.F.);
#93716=ADVANCED_FACE('',(#8743),#90542,.F.);
#93717=ADVANCED_FACE('',(#8744),#90543,.F.);
#93718=ADVANCED_FACE('',(#8745),#2554,.F.);
#93719=ADVANCED_FACE('',(#8746),#90544,.F.);
#93720=ADVANCED_FACE('',(#8747),#90545,.F.);
#93721=ADVANCED_FACE('',(#8748),#2555,.F.);
#93722=ADVANCED_FACE('',(#8749),#2556,.F.);
#93723=ADVANCED_FACE('',(#8750),#90546,.F.);
#93724=ADVANCED_FACE('',(#8751),#90547,.F.);
#93725=ADVANCED_FACE('',(#8752),#2557,.F.);
#93726=ADVANCED_FACE('',(#8753),#90548,.F.);
#93727=ADVANCED_FACE('',(#8754),#5798,.F.);
#93728=ADVANCED_FACE('',(#8755),#2558,.F.);
#93729=ADVANCED_FACE('',(#8756),#2559,.F.);
#93730=ADVANCED_FACE('',(#8757),#90549,.F.);
#93731=ADVANCED_FACE('',(#8758),#90550,.F.);
#93732=ADVANCED_FACE('',(#8759),#2560,.F.);
#93733=ADVANCED_FACE('',(#8760),#2561,.F.);
#93734=ADVANCED_FACE('',(#8761),#5799,.F.);
#93735=ADVANCED_FACE('',(#8762),#90551,.F.);
#93736=ADVANCED_FACE('',(#8763),#2562,.F.);
#93737=ADVANCED_FACE('',(#8764),#90552,.F.);
#93738=ADVANCED_FACE('',(#8765),#90553,.F.);
#93739=ADVANCED_FACE('',(#8766),#2563,.F.);
#93740=ADVANCED_FACE('',(#8767),#2564,.F.);
#93741=ADVANCED_FACE('',(#8768),#90554,.F.);
#93742=ADVANCED_FACE('',(#8769),#90555,.F.);
#93743=ADVANCED_FACE('',(#8770),#2565,.F.);
#93744=ADVANCED_FACE('',(#8771),#90556,.F.);
#93745=ADVANCED_FACE('',(#8772),#90557,.F.);
#93746=ADVANCED_FACE('',(#8773),#2566,.F.);
#93747=ADVANCED_FACE('',(#8774),#90558,.F.);
#93748=ADVANCED_FACE('',(#8775),#90559,.F.);
#93749=ADVANCED_FACE('',(#8776),#2567,.F.);
#93750=ADVANCED_FACE('',(#8777),#2568,.F.);
#93751=ADVANCED_FACE('',(#8778),#90560,.F.);
#93752=ADVANCED_FACE('',(#8779),#90561,.F.);
#93753=ADVANCED_FACE('',(#8780),#2569,.F.);
#93754=ADVANCED_FACE('',(#8781),#90562,.F.);
#93755=ADVANCED_FACE('',(#8782),#5800,.F.);
#93756=ADVANCED_FACE('',(#8783),#2570,.F.);
#93757=ADVANCED_FACE('',(#8784),#2571,.F.);
#93758=ADVANCED_FACE('',(#8785),#90563,.F.);
#93759=ADVANCED_FACE('',(#8786),#90564,.F.);
#93760=ADVANCED_FACE('',(#8787),#2572,.F.);
#93761=ADVANCED_FACE('',(#8788),#2573,.F.);
#93762=ADVANCED_FACE('',(#8789),#5801,.F.);
#93763=ADVANCED_FACE('',(#8790),#90565,.F.);
#93764=ADVANCED_FACE('',(#8791),#2574,.F.);
#93765=ADVANCED_FACE('',(#8792),#90566,.F.);
#93766=ADVANCED_FACE('',(#8793),#90567,.F.);
#93767=ADVANCED_FACE('',(#8794),#2575,.F.);
#93768=ADVANCED_FACE('',(#8795),#2576,.F.);
#93769=ADVANCED_FACE('',(#8796),#90568,.F.);
#93770=ADVANCED_FACE('',(#8797),#90569,.F.);
#93771=ADVANCED_FACE('',(#8798),#2577,.F.);
#93772=ADVANCED_FACE('',(#8799),#90570,.F.);
#93773=ADVANCED_FACE('',(#8800),#90571,.F.);
#93774=ADVANCED_FACE('',(#8801),#2578,.F.);
#93775=ADVANCED_FACE('',(#8802),#90572,.F.);
#93776=ADVANCED_FACE('',(#8803),#90573,.F.);
#93777=ADVANCED_FACE('',(#8804),#2579,.F.);
#93778=ADVANCED_FACE('',(#8805),#2580,.F.);
#93779=ADVANCED_FACE('',(#8806),#90574,.F.);
#93780=ADVANCED_FACE('',(#8807),#90575,.F.);
#93781=ADVANCED_FACE('',(#8808),#2581,.F.);
#93782=ADVANCED_FACE('',(#8809),#90576,.F.);
#93783=ADVANCED_FACE('',(#8810),#5802,.F.);
#93784=ADVANCED_FACE('',(#8811),#2582,.F.);
#93785=ADVANCED_FACE('',(#8812),#2583,.F.);
#93786=ADVANCED_FACE('',(#8813),#90577,.F.);
#93787=ADVANCED_FACE('',(#8814),#90578,.F.);
#93788=ADVANCED_FACE('',(#8815),#2584,.F.);
#93789=ADVANCED_FACE('',(#8816),#2585,.F.);
#93790=ADVANCED_FACE('',(#8817),#5803,.F.);
#93791=ADVANCED_FACE('',(#8818),#90579,.F.);
#93792=ADVANCED_FACE('',(#8819),#2586,.F.);
#93793=ADVANCED_FACE('',(#8820),#90580,.F.);
#93794=ADVANCED_FACE('',(#8821),#90581,.F.);
#93795=ADVANCED_FACE('',(#8822),#2587,.F.);
#93796=ADVANCED_FACE('',(#8823),#2588,.F.);
#93797=ADVANCED_FACE('',(#8824),#90582,.F.);
#93798=ADVANCED_FACE('',(#8825),#90583,.F.);
#93799=ADVANCED_FACE('',(#8826),#2589,.F.);
#93800=ADVANCED_FACE('',(#8827),#90584,.F.);
#93801=ADVANCED_FACE('',(#8828),#90585,.F.);
#93802=ADVANCED_FACE('',(#8829),#2590,.F.);
#93803=ADVANCED_FACE('',(#8830),#90586,.F.);
#93804=ADVANCED_FACE('',(#8831),#90587,.F.);
#93805=ADVANCED_FACE('',(#8832),#2591,.F.);
#93806=ADVANCED_FACE('',(#8833),#2592,.F.);
#93807=ADVANCED_FACE('',(#8834),#90588,.F.);
#93808=ADVANCED_FACE('',(#8835),#90589,.F.);
#93809=ADVANCED_FACE('',(#8836),#2593,.F.);
#93810=ADVANCED_FACE('',(#8837),#90590,.F.);
#93811=ADVANCED_FACE('',(#8838),#5804,.F.);
#93812=ADVANCED_FACE('',(#8839),#2594,.F.);
#93813=ADVANCED_FACE('',(#8840),#2595,.F.);
#93814=ADVANCED_FACE('',(#8841),#90591,.F.);
#93815=ADVANCED_FACE('',(#8842),#90592,.F.);
#93816=ADVANCED_FACE('',(#8843),#2596,.F.);
#93817=ADVANCED_FACE('',(#8844),#2597,.F.);
#93818=ADVANCED_FACE('',(#8845),#5805,.F.);
#93819=ADVANCED_FACE('',(#8846),#90593,.F.);
#93820=ADVANCED_FACE('',(#8847),#2598,.F.);
#93821=ADVANCED_FACE('',(#8848),#90594,.F.);
#93822=ADVANCED_FACE('',(#8849),#90595,.F.);
#93823=ADVANCED_FACE('',(#8850),#2599,.F.);
#93824=ADVANCED_FACE('',(#8851),#2600,.F.);
#93825=ADVANCED_FACE('',(#8852),#90596,.F.);
#93826=ADVANCED_FACE('',(#8853),#90597,.F.);
#93827=ADVANCED_FACE('',(#8854),#2601,.F.);
#93828=ADVANCED_FACE('',(#8855),#90598,.F.);
#93829=ADVANCED_FACE('',(#8856),#90599,.F.);
#93830=ADVANCED_FACE('',(#8857),#2602,.F.);
#93831=ADVANCED_FACE('',(#8858),#90600,.F.);
#93832=ADVANCED_FACE('',(#8859),#90601,.F.);
#93833=ADVANCED_FACE('',(#8860),#2603,.F.);
#93834=ADVANCED_FACE('',(#8861),#2604,.F.);
#93835=ADVANCED_FACE('',(#8862),#90602,.F.);
#93836=ADVANCED_FACE('',(#8863),#90603,.F.);
#93837=ADVANCED_FACE('',(#8864),#2605,.F.);
#93838=ADVANCED_FACE('',(#8865),#90604,.F.);
#93839=ADVANCED_FACE('',(#8866),#5806,.F.);
#93840=ADVANCED_FACE('',(#8867),#2606,.F.);
#93841=ADVANCED_FACE('',(#8868),#2607,.F.);
#93842=ADVANCED_FACE('',(#8869),#90605,.F.);
#93843=ADVANCED_FACE('',(#8870),#90606,.F.);
#93844=ADVANCED_FACE('',(#8871),#2608,.F.);
#93845=ADVANCED_FACE('',(#8872),#2609,.F.);
#93846=ADVANCED_FACE('',(#8873),#5807,.F.);
#93847=ADVANCED_FACE('',(#8874),#90607,.F.);
#93848=ADVANCED_FACE('',(#8875),#2610,.F.);
#93849=ADVANCED_FACE('',(#8876),#90608,.F.);
#93850=ADVANCED_FACE('',(#8877),#90609,.F.);
#93851=ADVANCED_FACE('',(#8878),#2611,.F.);
#93852=ADVANCED_FACE('',(#8879),#2612,.F.);
#93853=ADVANCED_FACE('',(#8880),#90610,.F.);
#93854=ADVANCED_FACE('',(#8881),#90611,.F.);
#93855=ADVANCED_FACE('',(#8882),#2613,.F.);
#93856=ADVANCED_FACE('',(#8883),#90612,.F.);
#93857=ADVANCED_FACE('',(#8884),#90613,.F.);
#93858=ADVANCED_FACE('',(#8885),#2614,.F.);
#93859=ADVANCED_FACE('',(#8886),#90614,.F.);
#93860=ADVANCED_FACE('',(#8887),#90615,.F.);
#93861=ADVANCED_FACE('',(#8888),#2615,.F.);
#93862=ADVANCED_FACE('',(#8889),#2616,.F.);
#93863=ADVANCED_FACE('',(#8890),#90616,.F.);
#93864=ADVANCED_FACE('',(#8891),#90617,.F.);
#93865=ADVANCED_FACE('',(#8892),#2617,.F.);
#93866=ADVANCED_FACE('',(#8893),#90618,.F.);
#93867=ADVANCED_FACE('',(#8894),#5808,.F.);
#93868=ADVANCED_FACE('',(#8895),#2618,.F.);
#93869=ADVANCED_FACE('',(#8896),#2619,.F.);
#93870=ADVANCED_FACE('',(#8897),#90619,.F.);
#93871=ADVANCED_FACE('',(#8898),#90620,.F.);
#93872=ADVANCED_FACE('',(#8899),#2620,.F.);
#93873=ADVANCED_FACE('',(#8900),#2621,.F.);
#93874=ADVANCED_FACE('',(#8901),#5809,.F.);
#93875=ADVANCED_FACE('',(#8902),#90621,.F.);
#93876=ADVANCED_FACE('',(#8903),#2622,.F.);
#93877=ADVANCED_FACE('',(#8904),#90622,.F.);
#93878=ADVANCED_FACE('',(#8905),#90623,.F.);
#93879=ADVANCED_FACE('',(#8906),#2623,.F.);
#93880=ADVANCED_FACE('',(#8907),#2624,.F.);
#93881=ADVANCED_FACE('',(#8908),#90624,.F.);
#93882=ADVANCED_FACE('',(#8909),#90625,.F.);
#93883=ADVANCED_FACE('',(#8910),#2625,.F.);
#93884=ADVANCED_FACE('',(#8911),#90626,.F.);
#93885=ADVANCED_FACE('',(#8912),#90627,.F.);
#93886=ADVANCED_FACE('',(#8913),#2626,.F.);
#93887=ADVANCED_FACE('',(#8914),#90628,.F.);
#93888=ADVANCED_FACE('',(#8915),#90629,.F.);
#93889=ADVANCED_FACE('',(#8916),#2627,.F.);
#93890=ADVANCED_FACE('',(#8917),#2628,.F.);
#93891=ADVANCED_FACE('',(#8918),#90630,.F.);
#93892=ADVANCED_FACE('',(#8919),#90631,.F.);
#93893=ADVANCED_FACE('',(#8920),#2629,.F.);
#93894=ADVANCED_FACE('',(#8921),#90632,.F.);
#93895=ADVANCED_FACE('',(#8922),#5810,.F.);
#93896=ADVANCED_FACE('',(#8923),#2630,.F.);
#93897=ADVANCED_FACE('',(#8924),#2631,.F.);
#93898=ADVANCED_FACE('',(#8925),#90633,.F.);
#93899=ADVANCED_FACE('',(#8926),#90634,.F.);
#93900=ADVANCED_FACE('',(#8927),#2632,.F.);
#93901=ADVANCED_FACE('',(#8928),#2633,.F.);
#93902=ADVANCED_FACE('',(#8929),#5811,.F.);
#93903=ADVANCED_FACE('',(#8930),#90635,.F.);
#93904=ADVANCED_FACE('',(#8931),#2634,.F.);
#93905=ADVANCED_FACE('',(#8932),#90636,.F.);
#93906=ADVANCED_FACE('',(#8933),#90637,.F.);
#93907=ADVANCED_FACE('',(#8934),#2635,.F.);
#93908=ADVANCED_FACE('',(#8935),#2636,.F.);
#93909=ADVANCED_FACE('',(#8936),#90638,.F.);
#93910=ADVANCED_FACE('',(#8937),#90639,.F.);
#93911=ADVANCED_FACE('',(#8938),#2637,.F.);
#93912=ADVANCED_FACE('',(#8939),#90640,.F.);
#93913=ADVANCED_FACE('',(#8940),#90641,.F.);
#93914=ADVANCED_FACE('',(#8941),#2638,.F.);
#93915=ADVANCED_FACE('',(#8942),#90642,.F.);
#93916=ADVANCED_FACE('',(#8943),#90643,.F.);
#93917=ADVANCED_FACE('',(#8944),#2639,.F.);
#93918=ADVANCED_FACE('',(#8945),#2640,.F.);
#93919=ADVANCED_FACE('',(#8946),#90644,.F.);
#93920=ADVANCED_FACE('',(#8947),#90645,.F.);
#93921=ADVANCED_FACE('',(#8948),#2641,.F.);
#93922=ADVANCED_FACE('',(#8949),#90646,.F.);
#93923=ADVANCED_FACE('',(#8950),#5812,.F.);
#93924=ADVANCED_FACE('',(#8951),#2642,.F.);
#93925=ADVANCED_FACE('',(#8952),#2643,.F.);
#93926=ADVANCED_FACE('',(#8953),#90647,.F.);
#93927=ADVANCED_FACE('',(#8954),#90648,.F.);
#93928=ADVANCED_FACE('',(#8955),#2644,.F.);
#93929=ADVANCED_FACE('',(#8956),#2645,.F.);
#93930=ADVANCED_FACE('',(#8957),#5813,.F.);
#93931=ADVANCED_FACE('',(#8958),#90649,.F.);
#93932=ADVANCED_FACE('',(#8959),#2646,.F.);
#93933=ADVANCED_FACE('',(#8960),#90650,.F.);
#93934=ADVANCED_FACE('',(#8961),#90651,.F.);
#93935=ADVANCED_FACE('',(#8962),#2647,.F.);
#93936=ADVANCED_FACE('',(#8963),#2648,.F.);
#93937=ADVANCED_FACE('',(#8964),#90652,.F.);
#93938=ADVANCED_FACE('',(#8965),#90653,.F.);
#93939=ADVANCED_FACE('',(#8966),#2649,.F.);
#93940=ADVANCED_FACE('',(#8967),#90654,.F.);
#93941=ADVANCED_FACE('',(#8968),#90655,.F.);
#93942=ADVANCED_FACE('',(#8969),#2650,.F.);
#93943=ADVANCED_FACE('',(#8970),#90656,.F.);
#93944=ADVANCED_FACE('',(#8971),#90657,.F.);
#93945=ADVANCED_FACE('',(#8972),#2651,.F.);
#93946=ADVANCED_FACE('',(#8973),#2652,.F.);
#93947=ADVANCED_FACE('',(#8974),#90658,.F.);
#93948=ADVANCED_FACE('',(#8975),#90659,.F.);
#93949=ADVANCED_FACE('',(#8976),#2653,.F.);
#93950=ADVANCED_FACE('',(#8977),#90660,.F.);
#93951=ADVANCED_FACE('',(#8978),#5814,.F.);
#93952=ADVANCED_FACE('',(#8979),#2654,.F.);
#93953=ADVANCED_FACE('',(#8980),#2655,.F.);
#93954=ADVANCED_FACE('',(#8981),#90661,.F.);
#93955=ADVANCED_FACE('',(#8982),#90662,.F.);
#93956=ADVANCED_FACE('',(#8983),#2656,.F.);
#93957=ADVANCED_FACE('',(#8984),#2657,.F.);
#93958=ADVANCED_FACE('',(#8985),#5815,.F.);
#93959=ADVANCED_FACE('',(#8986),#90663,.F.);
#93960=ADVANCED_FACE('',(#8987),#2658,.F.);
#93961=ADVANCED_FACE('',(#8988),#90664,.F.);
#93962=ADVANCED_FACE('',(#8989),#90665,.F.);
#93963=ADVANCED_FACE('',(#8990),#2659,.F.);
#93964=ADVANCED_FACE('',(#8991),#2660,.F.);
#93965=ADVANCED_FACE('',(#8992),#90666,.F.);
#93966=ADVANCED_FACE('',(#8993),#90667,.F.);
#93967=ADVANCED_FACE('',(#8994),#2661,.F.);
#93968=ADVANCED_FACE('',(#8995),#90668,.F.);
#93969=ADVANCED_FACE('',(#8996),#90669,.F.);
#93970=ADVANCED_FACE('',(#8997),#2662,.F.);
#93971=ADVANCED_FACE('',(#8998),#90670,.F.);
#93972=ADVANCED_FACE('',(#8999),#90671,.F.);
#93973=ADVANCED_FACE('',(#9000),#2663,.F.);
#93974=ADVANCED_FACE('',(#9001),#2664,.F.);
#93975=ADVANCED_FACE('',(#9002),#90672,.F.);
#93976=ADVANCED_FACE('',(#9003),#90673,.F.);
#93977=ADVANCED_FACE('',(#9004),#2665,.F.);
#93978=ADVANCED_FACE('',(#9005),#90674,.F.);
#93979=ADVANCED_FACE('',(#9006),#5816,.F.);
#93980=ADVANCED_FACE('',(#9007),#2666,.F.);
#93981=ADVANCED_FACE('',(#9008),#2667,.F.);
#93982=ADVANCED_FACE('',(#9009),#90675,.F.);
#93983=ADVANCED_FACE('',(#9010),#90676,.F.);
#93984=ADVANCED_FACE('',(#9011),#2668,.F.);
#93985=ADVANCED_FACE('',(#9012),#2669,.F.);
#93986=ADVANCED_FACE('',(#9013),#5817,.F.);
#93987=ADVANCED_FACE('',(#9014),#90677,.F.);
#93988=ADVANCED_FACE('',(#9015),#2670,.F.);
#93989=ADVANCED_FACE('',(#9016),#90678,.F.);
#93990=ADVANCED_FACE('',(#9017),#90679,.F.);
#93991=ADVANCED_FACE('',(#9018),#2671,.F.);
#93992=ADVANCED_FACE('',(#9019),#2672,.F.);
#93993=ADVANCED_FACE('',(#9020),#90680,.F.);
#93994=ADVANCED_FACE('',(#9021),#90681,.F.);
#93995=ADVANCED_FACE('',(#9022),#2673,.F.);
#93996=ADVANCED_FACE('',(#9023),#90682,.F.);
#93997=ADVANCED_FACE('',(#9024),#90683,.F.);
#93998=ADVANCED_FACE('',(#9025),#2674,.F.);
#93999=ADVANCED_FACE('',(#9026),#90684,.F.);
#94000=ADVANCED_FACE('',(#9027),#90685,.F.);
#94001=ADVANCED_FACE('',(#9028),#2675,.F.);
#94002=ADVANCED_FACE('',(#9029),#2676,.F.);
#94003=ADVANCED_FACE('',(#9030),#90686,.F.);
#94004=ADVANCED_FACE('',(#9031),#90687,.F.);
#94005=ADVANCED_FACE('',(#9032),#2677,.F.);
#94006=ADVANCED_FACE('',(#9033),#90688,.F.);
#94007=ADVANCED_FACE('',(#9034),#5818,.F.);
#94008=ADVANCED_FACE('',(#9035),#2678,.F.);
#94009=ADVANCED_FACE('',(#9036),#2679,.F.);
#94010=ADVANCED_FACE('',(#9037),#90689,.F.);
#94011=ADVANCED_FACE('',(#9038),#90690,.F.);
#94012=ADVANCED_FACE('',(#9039),#2680,.F.);
#94013=ADVANCED_FACE('',(#9040),#2681,.F.);
#94014=ADVANCED_FACE('',(#9041),#5819,.F.);
#94015=ADVANCED_FACE('',(#9042),#90691,.F.);
#94016=ADVANCED_FACE('',(#9043),#2682,.F.);
#94017=ADVANCED_FACE('',(#9044),#90692,.F.);
#94018=ADVANCED_FACE('',(#9045),#90693,.F.);
#94019=ADVANCED_FACE('',(#9046),#2683,.F.);
#94020=ADVANCED_FACE('',(#9047),#2684,.F.);
#94021=ADVANCED_FACE('',(#9048),#90694,.F.);
#94022=ADVANCED_FACE('',(#9049),#90695,.F.);
#94023=ADVANCED_FACE('',(#9050),#2685,.F.);
#94024=ADVANCED_FACE('',(#9051),#90696,.F.);
#94025=ADVANCED_FACE('',(#9052),#90697,.F.);
#94026=ADVANCED_FACE('',(#9053),#2686,.F.);
#94027=ADVANCED_FACE('',(#9054),#90698,.F.);
#94028=ADVANCED_FACE('',(#9055),#90699,.F.);
#94029=ADVANCED_FACE('',(#9056),#2687,.F.);
#94030=ADVANCED_FACE('',(#9057),#2688,.F.);
#94031=ADVANCED_FACE('',(#9058),#90700,.F.);
#94032=ADVANCED_FACE('',(#9059),#90701,.F.);
#94033=ADVANCED_FACE('',(#9060),#2689,.F.);
#94034=ADVANCED_FACE('',(#9061),#90702,.F.);
#94035=ADVANCED_FACE('',(#9062),#5820,.F.);
#94036=ADVANCED_FACE('',(#9063),#2690,.F.);
#94037=ADVANCED_FACE('',(#9064),#2691,.F.);
#94038=ADVANCED_FACE('',(#9065),#90703,.F.);
#94039=ADVANCED_FACE('',(#9066),#90704,.F.);
#94040=ADVANCED_FACE('',(#9067),#2692,.F.);
#94041=ADVANCED_FACE('',(#9068),#2693,.F.);
#94042=ADVANCED_FACE('',(#9069),#5821,.F.);
#94043=ADVANCED_FACE('',(#9070),#90705,.F.);
#94044=ADVANCED_FACE('',(#9071),#2694,.F.);
#94045=ADVANCED_FACE('',(#9072),#90706,.F.);
#94046=ADVANCED_FACE('',(#9073),#90707,.F.);
#94047=ADVANCED_FACE('',(#9074),#2695,.F.);
#94048=ADVANCED_FACE('',(#9075),#2696,.F.);
#94049=ADVANCED_FACE('',(#9076),#90708,.F.);
#94050=ADVANCED_FACE('',(#9077),#90709,.F.);
#94051=ADVANCED_FACE('',(#9078),#2697,.F.);
#94052=ADVANCED_FACE('',(#9079),#90710,.F.);
#94053=ADVANCED_FACE('',(#9080),#90711,.F.);
#94054=ADVANCED_FACE('',(#9081),#2698,.F.);
#94055=ADVANCED_FACE('',(#9082),#90712,.F.);
#94056=ADVANCED_FACE('',(#9083),#90713,.F.);
#94057=ADVANCED_FACE('',(#9084),#2699,.F.);
#94058=ADVANCED_FACE('',(#9085),#2700,.F.);
#94059=ADVANCED_FACE('',(#9086),#90714,.F.);
#94060=ADVANCED_FACE('',(#9087),#90715,.F.);
#94061=ADVANCED_FACE('',(#9088),#2701,.F.);
#94062=ADVANCED_FACE('',(#9089),#90716,.F.);
#94063=ADVANCED_FACE('',(#9090),#5822,.F.);
#94064=ADVANCED_FACE('',(#9091),#2702,.F.);
#94065=ADVANCED_FACE('',(#9092),#2703,.F.);
#94066=ADVANCED_FACE('',(#9093),#90717,.F.);
#94067=ADVANCED_FACE('',(#9094),#90718,.F.);
#94068=ADVANCED_FACE('',(#9095),#2704,.F.);
#94069=ADVANCED_FACE('',(#9096),#2705,.F.);
#94070=ADVANCED_FACE('',(#9097),#5823,.F.);
#94071=ADVANCED_FACE('',(#9098),#90719,.F.);
#94072=ADVANCED_FACE('',(#9099),#2706,.F.);
#94073=ADVANCED_FACE('',(#9100),#90720,.F.);
#94074=ADVANCED_FACE('',(#9101),#90721,.F.);
#94075=ADVANCED_FACE('',(#9102),#2707,.F.);
#94076=ADVANCED_FACE('',(#9103),#2708,.F.);
#94077=ADVANCED_FACE('',(#9104),#90722,.F.);
#94078=ADVANCED_FACE('',(#9105),#90723,.F.);
#94079=ADVANCED_FACE('',(#9106),#2709,.F.);
#94080=ADVANCED_FACE('',(#9107),#90724,.F.);
#94081=ADVANCED_FACE('',(#9108),#90725,.F.);
#94082=ADVANCED_FACE('',(#9109),#2710,.F.);
#94083=ADVANCED_FACE('',(#9110),#90726,.F.);
#94084=ADVANCED_FACE('',(#9111),#90727,.F.);
#94085=ADVANCED_FACE('',(#9112),#2711,.F.);
#94086=ADVANCED_FACE('',(#9113),#2712,.F.);
#94087=ADVANCED_FACE('',(#9114),#90728,.F.);
#94088=ADVANCED_FACE('',(#9115),#90729,.F.);
#94089=ADVANCED_FACE('',(#9116),#2713,.F.);
#94090=ADVANCED_FACE('',(#9117),#90730,.F.);
#94091=ADVANCED_FACE('',(#9118),#5824,.F.);
#94092=ADVANCED_FACE('',(#9119),#2714,.F.);
#94093=ADVANCED_FACE('',(#9120),#2715,.F.);
#94094=ADVANCED_FACE('',(#9121),#90731,.F.);
#94095=ADVANCED_FACE('',(#9122),#90732,.F.);
#94096=ADVANCED_FACE('',(#9123),#2716,.F.);
#94097=ADVANCED_FACE('',(#9124),#2717,.F.);
#94098=ADVANCED_FACE('',(#9125),#5825,.F.);
#94099=ADVANCED_FACE('',(#9126),#90733,.F.);
#94100=ADVANCED_FACE('',(#9127),#2718,.F.);
#94101=ADVANCED_FACE('',(#9128),#90734,.F.);
#94102=ADVANCED_FACE('',(#9129),#90735,.F.);
#94103=ADVANCED_FACE('',(#9130),#2719,.F.);
#94104=ADVANCED_FACE('',(#9131),#2720,.F.);
#94105=ADVANCED_FACE('',(#9132),#90736,.F.);
#94106=ADVANCED_FACE('',(#9133),#90737,.F.);
#94107=ADVANCED_FACE('',(#9134),#2721,.F.);
#94108=ADVANCED_FACE('',(#9135),#90738,.F.);
#94109=ADVANCED_FACE('',(#9136),#90739,.F.);
#94110=ADVANCED_FACE('',(#9137),#2722,.F.);
#94111=ADVANCED_FACE('',(#9138),#90740,.F.);
#94112=ADVANCED_FACE('',(#9139),#90741,.F.);
#94113=ADVANCED_FACE('',(#9140),#2723,.F.);
#94114=ADVANCED_FACE('',(#9141),#2724,.F.);
#94115=ADVANCED_FACE('',(#9142),#90742,.F.);
#94116=ADVANCED_FACE('',(#9143),#90743,.F.);
#94117=ADVANCED_FACE('',(#9144),#2725,.F.);
#94118=ADVANCED_FACE('',(#9145),#90744,.F.);
#94119=ADVANCED_FACE('',(#9146),#5826,.F.);
#94120=ADVANCED_FACE('',(#9147),#2726,.F.);
#94121=ADVANCED_FACE('',(#9148),#2727,.F.);
#94122=ADVANCED_FACE('',(#9149),#90745,.F.);
#94123=ADVANCED_FACE('',(#9150),#90746,.F.);
#94124=ADVANCED_FACE('',(#9151),#2728,.F.);
#94125=ADVANCED_FACE('',(#9152),#2729,.F.);
#94126=ADVANCED_FACE('',(#9153),#5827,.F.);
#94127=ADVANCED_FACE('',(#9154),#90747,.F.);
#94128=ADVANCED_FACE('',(#9155),#2730,.F.);
#94129=ADVANCED_FACE('',(#9156),#90748,.F.);
#94130=ADVANCED_FACE('',(#9157),#90749,.F.);
#94131=ADVANCED_FACE('',(#9158),#2731,.F.);
#94132=ADVANCED_FACE('',(#9159),#2732,.F.);
#94133=ADVANCED_FACE('',(#9160),#90750,.F.);
#94134=ADVANCED_FACE('',(#9161),#90751,.F.);
#94135=ADVANCED_FACE('',(#9162),#2733,.F.);
#94136=ADVANCED_FACE('',(#9163),#90752,.F.);
#94137=ADVANCED_FACE('',(#9164),#90753,.F.);
#94138=ADVANCED_FACE('',(#9165),#2734,.F.);
#94139=ADVANCED_FACE('',(#9166),#90754,.F.);
#94140=ADVANCED_FACE('',(#9167),#90755,.F.);
#94141=ADVANCED_FACE('',(#9168),#2735,.F.);
#94142=ADVANCED_FACE('',(#9169),#2736,.F.);
#94143=ADVANCED_FACE('',(#9170),#90756,.F.);
#94144=ADVANCED_FACE('',(#9171),#90757,.F.);
#94145=ADVANCED_FACE('',(#9172),#2737,.F.);
#94146=ADVANCED_FACE('',(#9173),#90758,.F.);
#94147=ADVANCED_FACE('',(#9174),#5828,.F.);
#94148=ADVANCED_FACE('',(#9175),#2738,.F.);
#94149=ADVANCED_FACE('',(#9176),#2739,.F.);
#94150=ADVANCED_FACE('',(#9177),#90759,.F.);
#94151=ADVANCED_FACE('',(#9178),#90760,.F.);
#94152=ADVANCED_FACE('',(#9179),#2740,.F.);
#94153=ADVANCED_FACE('',(#9180),#2741,.F.);
#94154=ADVANCED_FACE('',(#9181),#5829,.F.);
#94155=ADVANCED_FACE('',(#9182),#90761,.F.);
#94156=ADVANCED_FACE('',(#9183),#2742,.F.);
#94157=ADVANCED_FACE('',(#9184),#90762,.F.);
#94158=ADVANCED_FACE('',(#9185),#90763,.F.);
#94159=ADVANCED_FACE('',(#9186),#2743,.F.);
#94160=ADVANCED_FACE('',(#9187),#2744,.F.);
#94161=ADVANCED_FACE('',(#9188),#90764,.F.);
#94162=ADVANCED_FACE('',(#9189),#90765,.F.);
#94163=ADVANCED_FACE('',(#9190),#2745,.F.);
#94164=ADVANCED_FACE('',(#9191),#90766,.F.);
#94165=ADVANCED_FACE('',(#9192),#90767,.F.);
#94166=ADVANCED_FACE('',(#9193),#2746,.F.);
#94167=ADVANCED_FACE('',(#9194),#90768,.F.);
#94168=ADVANCED_FACE('',(#9195),#90769,.F.);
#94169=ADVANCED_FACE('',(#9196),#2747,.F.);
#94170=ADVANCED_FACE('',(#9197),#2748,.F.);
#94171=ADVANCED_FACE('',(#9198),#90770,.F.);
#94172=ADVANCED_FACE('',(#9199),#90771,.F.);
#94173=ADVANCED_FACE('',(#9200),#2749,.F.);
#94174=ADVANCED_FACE('',(#9201),#90772,.F.);
#94175=ADVANCED_FACE('',(#9202),#5830,.F.);
#94176=ADVANCED_FACE('',(#9203),#2750,.F.);
#94177=ADVANCED_FACE('',(#9204),#2751,.F.);
#94178=ADVANCED_FACE('',(#9205),#90773,.F.);
#94179=ADVANCED_FACE('',(#9206),#90774,.F.);
#94180=ADVANCED_FACE('',(#9207),#2752,.F.);
#94181=ADVANCED_FACE('',(#9208),#2753,.F.);
#94182=ADVANCED_FACE('',(#9209),#5831,.F.);
#94183=ADVANCED_FACE('',(#9210),#90775,.F.);
#94184=ADVANCED_FACE('',(#9211),#2754,.F.);
#94185=ADVANCED_FACE('',(#9212),#90776,.F.);
#94186=ADVANCED_FACE('',(#9213),#90777,.F.);
#94187=ADVANCED_FACE('',(#9214),#2755,.F.);
#94188=ADVANCED_FACE('',(#9215),#2756,.F.);
#94189=ADVANCED_FACE('',(#9216),#90778,.F.);
#94190=ADVANCED_FACE('',(#9217),#90779,.F.);
#94191=ADVANCED_FACE('',(#9218),#2757,.F.);
#94192=ADVANCED_FACE('',(#9219),#90780,.F.);
#94193=ADVANCED_FACE('',(#9220),#90781,.F.);
#94194=ADVANCED_FACE('',(#9221),#2758,.F.);
#94195=ADVANCED_FACE('',(#9222),#90782,.F.);
#94196=ADVANCED_FACE('',(#9223),#90783,.F.);
#94197=ADVANCED_FACE('',(#9224),#2759,.F.);
#94198=ADVANCED_FACE('',(#9225),#2760,.F.);
#94199=ADVANCED_FACE('',(#9226),#90784,.F.);
#94200=ADVANCED_FACE('',(#9227),#90785,.F.);
#94201=ADVANCED_FACE('',(#9228),#2761,.F.);
#94202=ADVANCED_FACE('',(#9229),#90786,.F.);
#94203=ADVANCED_FACE('',(#9230),#5832,.F.);
#94204=ADVANCED_FACE('',(#9231),#2762,.F.);
#94205=ADVANCED_FACE('',(#9232),#2763,.F.);
#94206=ADVANCED_FACE('',(#9233),#90787,.F.);
#94207=ADVANCED_FACE('',(#9234),#90788,.F.);
#94208=ADVANCED_FACE('',(#9235),#2764,.F.);
#94209=ADVANCED_FACE('',(#9236),#2765,.F.);
#94210=ADVANCED_FACE('',(#9237),#5833,.F.);
#94211=ADVANCED_FACE('',(#9238),#90789,.F.);
#94212=ADVANCED_FACE('',(#9239),#2766,.F.);
#94213=ADVANCED_FACE('',(#9240),#90790,.F.);
#94214=ADVANCED_FACE('',(#9241),#90791,.F.);
#94215=ADVANCED_FACE('',(#9242),#2767,.F.);
#94216=ADVANCED_FACE('',(#9243),#2768,.F.);
#94217=ADVANCED_FACE('',(#9244),#90792,.F.);
#94218=ADVANCED_FACE('',(#9245),#90793,.F.);
#94219=ADVANCED_FACE('',(#9246),#2769,.F.);
#94220=ADVANCED_FACE('',(#9247),#90794,.F.);
#94221=ADVANCED_FACE('',(#9248),#90795,.F.);
#94222=ADVANCED_FACE('',(#9249),#2770,.F.);
#94223=ADVANCED_FACE('',(#9250),#90796,.F.);
#94224=ADVANCED_FACE('',(#9251),#90797,.F.);
#94225=ADVANCED_FACE('',(#9252),#2771,.F.);
#94226=ADVANCED_FACE('',(#9253),#2772,.F.);
#94227=ADVANCED_FACE('',(#9254),#90798,.F.);
#94228=ADVANCED_FACE('',(#9255),#90799,.F.);
#94229=ADVANCED_FACE('',(#9256),#2773,.F.);
#94230=ADVANCED_FACE('',(#9257),#90800,.F.);
#94231=ADVANCED_FACE('',(#9258),#5834,.F.);
#94232=ADVANCED_FACE('',(#9259),#2774,.F.);
#94233=ADVANCED_FACE('',(#9260),#2775,.F.);
#94234=ADVANCED_FACE('',(#9261),#90801,.F.);
#94235=ADVANCED_FACE('',(#9262),#90802,.F.);
#94236=ADVANCED_FACE('',(#9263),#2776,.F.);
#94237=ADVANCED_FACE('',(#9264),#2777,.F.);
#94238=ADVANCED_FACE('',(#9265),#5835,.F.);
#94239=ADVANCED_FACE('',(#9266),#90803,.F.);
#94240=ADVANCED_FACE('',(#9267),#2778,.F.);
#94241=ADVANCED_FACE('',(#9268),#90804,.F.);
#94242=ADVANCED_FACE('',(#9269),#90805,.F.);
#94243=ADVANCED_FACE('',(#9270),#2779,.F.);
#94244=ADVANCED_FACE('',(#9271),#2780,.F.);
#94245=ADVANCED_FACE('',(#9272),#90806,.F.);
#94246=ADVANCED_FACE('',(#9273),#90807,.F.);
#94247=ADVANCED_FACE('',(#9274),#2781,.F.);
#94248=ADVANCED_FACE('',(#9275),#90808,.F.);
#94249=ADVANCED_FACE('',(#9276),#90809,.F.);
#94250=ADVANCED_FACE('',(#9277),#2782,.F.);
#94251=ADVANCED_FACE('',(#9278),#90810,.F.);
#94252=ADVANCED_FACE('',(#9279),#90811,.F.);
#94253=ADVANCED_FACE('',(#9280),#2783,.F.);
#94254=ADVANCED_FACE('',(#9281),#2784,.F.);
#94255=ADVANCED_FACE('',(#9282),#90812,.F.);
#94256=ADVANCED_FACE('',(#9283),#90813,.F.);
#94257=ADVANCED_FACE('',(#9284),#2785,.F.);
#94258=ADVANCED_FACE('',(#9285),#90814,.F.);
#94259=ADVANCED_FACE('',(#9286),#5836,.F.);
#94260=ADVANCED_FACE('',(#9287),#2786,.F.);
#94261=ADVANCED_FACE('',(#9288),#2787,.F.);
#94262=ADVANCED_FACE('',(#9289),#90815,.F.);
#94263=ADVANCED_FACE('',(#9290),#90816,.F.);
#94264=ADVANCED_FACE('',(#9291),#2788,.F.);
#94265=ADVANCED_FACE('',(#9292),#2789,.F.);
#94266=ADVANCED_FACE('',(#9293),#5837,.F.);
#94267=ADVANCED_FACE('',(#9294),#90817,.F.);
#94268=ADVANCED_FACE('',(#9295),#2790,.F.);
#94269=ADVANCED_FACE('',(#9296),#90818,.F.);
#94270=ADVANCED_FACE('',(#9297),#90819,.F.);
#94271=ADVANCED_FACE('',(#9298),#2791,.F.);
#94272=ADVANCED_FACE('',(#9299),#2792,.F.);
#94273=ADVANCED_FACE('',(#9300),#90820,.F.);
#94274=ADVANCED_FACE('',(#9301),#90821,.F.);
#94275=ADVANCED_FACE('',(#9302),#2793,.F.);
#94276=ADVANCED_FACE('',(#9303),#90822,.F.);
#94277=ADVANCED_FACE('',(#9304),#90823,.F.);
#94278=ADVANCED_FACE('',(#9305),#2794,.F.);
#94279=ADVANCED_FACE('',(#9306),#90824,.F.);
#94280=ADVANCED_FACE('',(#9307),#90825,.F.);
#94281=ADVANCED_FACE('',(#9308),#2795,.F.);
#94282=ADVANCED_FACE('',(#9309),#2796,.F.);
#94283=ADVANCED_FACE('',(#9310),#90826,.F.);
#94284=ADVANCED_FACE('',(#9311),#90827,.F.);
#94285=ADVANCED_FACE('',(#9312),#2797,.F.);
#94286=ADVANCED_FACE('',(#9313),#90828,.F.);
#94287=ADVANCED_FACE('',(#9314),#5838,.F.);
#94288=ADVANCED_FACE('',(#9315),#2798,.F.);
#94289=ADVANCED_FACE('',(#9316),#2799,.F.);
#94290=ADVANCED_FACE('',(#9317),#90829,.F.);
#94291=ADVANCED_FACE('',(#9318),#90830,.F.);
#94292=ADVANCED_FACE('',(#9319),#2800,.F.);
#94293=ADVANCED_FACE('',(#9320),#2801,.F.);
#94294=ADVANCED_FACE('',(#9321),#5839,.F.);
#94295=ADVANCED_FACE('',(#9322),#90831,.F.);
#94296=ADVANCED_FACE('',(#9323),#2802,.F.);
#94297=ADVANCED_FACE('',(#9324),#90832,.F.);
#94298=ADVANCED_FACE('',(#9325),#90833,.F.);
#94299=ADVANCED_FACE('',(#9326),#2803,.F.);
#94300=ADVANCED_FACE('',(#9327),#2804,.F.);
#94301=ADVANCED_FACE('',(#9328),#90834,.F.);
#94302=ADVANCED_FACE('',(#9329),#90835,.F.);
#94303=ADVANCED_FACE('',(#9330),#2805,.F.);
#94304=ADVANCED_FACE('',(#9331),#90836,.F.);
#94305=ADVANCED_FACE('',(#9332),#90837,.F.);
#94306=ADVANCED_FACE('',(#9333),#2806,.F.);
#94307=ADVANCED_FACE('',(#9334),#90838,.F.);
#94308=ADVANCED_FACE('',(#9335),#90839,.F.);
#94309=ADVANCED_FACE('',(#9336),#2807,.F.);
#94310=ADVANCED_FACE('',(#9337),#2808,.F.);
#94311=ADVANCED_FACE('',(#9338),#90840,.F.);
#94312=ADVANCED_FACE('',(#9339),#90841,.F.);
#94313=ADVANCED_FACE('',(#9340),#2809,.F.);
#94314=ADVANCED_FACE('',(#9341),#90842,.F.);
#94315=ADVANCED_FACE('',(#9342),#5840,.F.);
#94316=ADVANCED_FACE('',(#9343),#2810,.F.);
#94317=ADVANCED_FACE('',(#9344),#2811,.F.);
#94318=ADVANCED_FACE('',(#9345),#90843,.F.);
#94319=ADVANCED_FACE('',(#9346),#90844,.F.);
#94320=ADVANCED_FACE('',(#9347),#2812,.F.);
#94321=ADVANCED_FACE('',(#9348),#2813,.F.);
#94322=ADVANCED_FACE('',(#9349),#5841,.F.);
#94323=ADVANCED_FACE('',(#9350),#90845,.F.);
#94324=ADVANCED_FACE('',(#9351),#2814,.F.);
#94325=ADVANCED_FACE('',(#9352),#90846,.F.);
#94326=ADVANCED_FACE('',(#9353),#90847,.F.);
#94327=ADVANCED_FACE('',(#9354),#2815,.F.);
#94328=ADVANCED_FACE('',(#9355),#2816,.F.);
#94329=ADVANCED_FACE('',(#9356),#90848,.F.);
#94330=ADVANCED_FACE('',(#9357),#90849,.F.);
#94331=ADVANCED_FACE('',(#9358),#2817,.F.);
#94332=ADVANCED_FACE('',(#9359),#90850,.F.);
#94333=ADVANCED_FACE('',(#9360),#90851,.F.);
#94334=ADVANCED_FACE('',(#9361),#2818,.F.);
#94335=ADVANCED_FACE('',(#9362),#90852,.F.);
#94336=ADVANCED_FACE('',(#9363),#90853,.F.);
#94337=ADVANCED_FACE('',(#9364),#2819,.F.);
#94338=ADVANCED_FACE('',(#9365),#2820,.F.);
#94339=ADVANCED_FACE('',(#9366),#90854,.F.);
#94340=ADVANCED_FACE('',(#9367),#90855,.F.);
#94341=ADVANCED_FACE('',(#9368),#2821,.F.);
#94342=ADVANCED_FACE('',(#9369),#90856,.F.);
#94343=ADVANCED_FACE('',(#9370),#5842,.F.);
#94344=ADVANCED_FACE('',(#9371),#2822,.F.);
#94345=ADVANCED_FACE('',(#9372),#2823,.F.);
#94346=ADVANCED_FACE('',(#9373),#90857,.F.);
#94347=ADVANCED_FACE('',(#9374),#90858,.F.);
#94348=ADVANCED_FACE('',(#9375),#2824,.F.);
#94349=ADVANCED_FACE('',(#9376),#2825,.F.);
#94350=ADVANCED_FACE('',(#9377),#5843,.F.);
#94351=ADVANCED_FACE('',(#9378),#90859,.F.);
#94352=ADVANCED_FACE('',(#9379),#2826,.F.);
#94353=ADVANCED_FACE('',(#9380),#90860,.F.);
#94354=ADVANCED_FACE('',(#9381),#90861,.F.);
#94355=ADVANCED_FACE('',(#9382),#2827,.F.);
#94356=ADVANCED_FACE('',(#9383),#2828,.F.);
#94357=ADVANCED_FACE('',(#9384),#90862,.F.);
#94358=ADVANCED_FACE('',(#9385),#90863,.F.);
#94359=ADVANCED_FACE('',(#9386),#2829,.F.);
#94360=ADVANCED_FACE('',(#9387),#90864,.F.);
#94361=ADVANCED_FACE('',(#9388),#90865,.F.);
#94362=ADVANCED_FACE('',(#9389),#2830,.F.);
#94363=ADVANCED_FACE('',(#9390),#90866,.F.);
#94364=ADVANCED_FACE('',(#9391),#90867,.F.);
#94365=ADVANCED_FACE('',(#9392),#2831,.F.);
#94366=ADVANCED_FACE('',(#9393),#2832,.F.);
#94367=ADVANCED_FACE('',(#9394),#90868,.F.);
#94368=ADVANCED_FACE('',(#9395),#90869,.F.);
#94369=ADVANCED_FACE('',(#9396),#2833,.F.);
#94370=ADVANCED_FACE('',(#9397),#90870,.F.);
#94371=ADVANCED_FACE('',(#9398),#5844,.F.);
#94372=ADVANCED_FACE('',(#9399),#2834,.F.);
#94373=ADVANCED_FACE('',(#9400),#2835,.F.);
#94374=ADVANCED_FACE('',(#9401),#90871,.F.);
#94375=ADVANCED_FACE('',(#9402),#90872,.F.);
#94376=ADVANCED_FACE('',(#9403),#2836,.F.);
#94377=ADVANCED_FACE('',(#9404),#2837,.F.);
#94378=ADVANCED_FACE('',(#9405),#5845,.F.);
#94379=ADVANCED_FACE('',(#9406),#90873,.F.);
#94380=ADVANCED_FACE('',(#9407),#2838,.F.);
#94381=ADVANCED_FACE('',(#9408),#90874,.F.);
#94382=ADVANCED_FACE('',(#9409),#90875,.F.);
#94383=ADVANCED_FACE('',(#9410),#2839,.F.);
#94384=ADVANCED_FACE('',(#9411),#2840,.F.);
#94385=ADVANCED_FACE('',(#9412),#90876,.F.);
#94386=ADVANCED_FACE('',(#9413),#90877,.F.);
#94387=ADVANCED_FACE('',(#9414),#2841,.F.);
#94388=ADVANCED_FACE('',(#9415),#90878,.F.);
#94389=ADVANCED_FACE('',(#9416),#90879,.F.);
#94390=ADVANCED_FACE('',(#9417),#2842,.F.);
#94391=ADVANCED_FACE('',(#9418),#90880,.F.);
#94392=ADVANCED_FACE('',(#9419),#90881,.F.);
#94393=ADVANCED_FACE('',(#9420),#2843,.F.);
#94394=ADVANCED_FACE('',(#9421),#2844,.F.);
#94395=ADVANCED_FACE('',(#9422),#90882,.F.);
#94396=ADVANCED_FACE('',(#9423),#90883,.F.);
#94397=ADVANCED_FACE('',(#9424),#2845,.F.);
#94398=ADVANCED_FACE('',(#9425),#90884,.F.);
#94399=ADVANCED_FACE('',(#9426),#5846,.F.);
#94400=ADVANCED_FACE('',(#9427),#2846,.F.);
#94401=ADVANCED_FACE('',(#9428),#2847,.F.);
#94402=ADVANCED_FACE('',(#9429),#90885,.F.);
#94403=ADVANCED_FACE('',(#9430),#90886,.F.);
#94404=ADVANCED_FACE('',(#9431),#2848,.F.);
#94405=ADVANCED_FACE('',(#9432),#2849,.F.);
#94406=ADVANCED_FACE('',(#9433),#5847,.F.);
#94407=ADVANCED_FACE('',(#9434),#90887,.F.);
#94408=ADVANCED_FACE('',(#9435),#2850,.F.);
#94409=ADVANCED_FACE('',(#9436),#90888,.F.);
#94410=ADVANCED_FACE('',(#9437),#90889,.F.);
#94411=ADVANCED_FACE('',(#9438),#2851,.F.);
#94412=ADVANCED_FACE('',(#9439),#2852,.F.);
#94413=ADVANCED_FACE('',(#9440),#90890,.F.);
#94414=ADVANCED_FACE('',(#9441),#90891,.F.);
#94415=ADVANCED_FACE('',(#9442),#2853,.F.);
#94416=ADVANCED_FACE('',(#9443),#90892,.F.);
#94417=ADVANCED_FACE('',(#9444),#90893,.F.);
#94418=ADVANCED_FACE('',(#9445),#2854,.F.);
#94419=ADVANCED_FACE('',(#9446),#90894,.F.);
#94420=ADVANCED_FACE('',(#9447),#90895,.F.);
#94421=ADVANCED_FACE('',(#9448),#2855,.F.);
#94422=ADVANCED_FACE('',(#9449),#2856,.F.);
#94423=ADVANCED_FACE('',(#9450),#90896,.F.);
#94424=ADVANCED_FACE('',(#9451),#90897,.F.);
#94425=ADVANCED_FACE('',(#9452),#2857,.F.);
#94426=ADVANCED_FACE('',(#9453),#90898,.F.);
#94427=ADVANCED_FACE('',(#9454),#5848,.F.);
#94428=ADVANCED_FACE('',(#9455),#2858,.F.);
#94429=ADVANCED_FACE('',(#9456),#2859,.F.);
#94430=ADVANCED_FACE('',(#9457),#90899,.F.);
#94431=ADVANCED_FACE('',(#9458),#90900,.F.);
#94432=ADVANCED_FACE('',(#9459),#2860,.F.);
#94433=ADVANCED_FACE('',(#9460),#2861,.F.);
#94434=ADVANCED_FACE('',(#9461),#5849,.F.);
#94435=ADVANCED_FACE('',(#9462),#90901,.F.);
#94436=ADVANCED_FACE('',(#9463),#2862,.F.);
#94437=ADVANCED_FACE('',(#9464),#90902,.F.);
#94438=ADVANCED_FACE('',(#9465),#90903,.F.);
#94439=ADVANCED_FACE('',(#9466),#2863,.F.);
#94440=ADVANCED_FACE('',(#9467),#2864,.F.);
#94441=ADVANCED_FACE('',(#9468),#90904,.F.);
#94442=ADVANCED_FACE('',(#9469),#90905,.F.);
#94443=ADVANCED_FACE('',(#9470),#2865,.F.);
#94444=ADVANCED_FACE('',(#9471),#90906,.F.);
#94445=ADVANCED_FACE('',(#9472),#90907,.F.);
#94446=ADVANCED_FACE('',(#9473),#2866,.F.);
#94447=ADVANCED_FACE('',(#9474),#90908,.F.);
#94448=ADVANCED_FACE('',(#9475),#90909,.F.);
#94449=ADVANCED_FACE('',(#9476),#2867,.F.);
#94450=ADVANCED_FACE('',(#9477),#2868,.F.);
#94451=ADVANCED_FACE('',(#9478),#90910,.F.);
#94452=ADVANCED_FACE('',(#9479),#90911,.F.);
#94453=ADVANCED_FACE('',(#9480),#2869,.F.);
#94454=ADVANCED_FACE('',(#9481),#90912,.F.);
#94455=ADVANCED_FACE('',(#9482),#2870,.F.);
#94456=ADVANCED_FACE('',(#9483),#2871,.F.);
#94457=ADVANCED_FACE('',(#9484),#90913,.F.);
#94458=ADVANCED_FACE('',(#9485),#90914,.F.);
#94459=ADVANCED_FACE('',(#9486),#2872,.F.);
#94460=ADVANCED_FACE('',(#9487),#2873,.F.);
#94461=ADVANCED_FACE('',(#9488),#90915,.F.);
#94462=ADVANCED_FACE('',(#9489),#2874,.F.);
#94463=ADVANCED_FACE('',(#9490),#90916,.F.);
#94464=ADVANCED_FACE('',(#9491),#90917,.F.);
#94465=ADVANCED_FACE('',(#9492),#2875,.F.);
#94466=ADVANCED_FACE('',(#9493),#2876,.F.);
#94467=ADVANCED_FACE('',(#9494),#90918,.F.);
#94468=ADVANCED_FACE('',(#9495),#90919,.F.);
#94469=ADVANCED_FACE('',(#9496),#2877,.F.);
#94470=ADVANCED_FACE('',(#9497),#90920,.F.);
#94471=ADVANCED_FACE('',(#9498),#90921,.F.);
#94472=ADVANCED_FACE('',(#9499),#2878,.F.);
#94473=ADVANCED_FACE('',(#9500),#90922,.F.);
#94474=ADVANCED_FACE('',(#9501),#90923,.F.);
#94475=ADVANCED_FACE('',(#9502),#2879,.F.);
#94476=ADVANCED_FACE('',(#9503),#2880,.F.);
#94477=ADVANCED_FACE('',(#9504),#90924,.F.);
#94478=ADVANCED_FACE('',(#9505),#90925,.F.);
#94479=ADVANCED_FACE('',(#9506),#2881,.F.);
#94480=ADVANCED_FACE('',(#9507),#90926,.F.);
#94481=ADVANCED_FACE('',(#9508),#5850,.F.);
#94482=ADVANCED_FACE('',(#9509),#2882,.F.);
#94483=ADVANCED_FACE('',(#9510),#2883,.F.);
#94484=ADVANCED_FACE('',(#9511),#90927,.F.);
#94485=ADVANCED_FACE('',(#9512),#90928,.F.);
#94486=ADVANCED_FACE('',(#9513),#2884,.F.);
#94487=ADVANCED_FACE('',(#9514),#2885,.F.);
#94488=ADVANCED_FACE('',(#9515),#5851,.F.);
#94489=ADVANCED_FACE('',(#9516),#90929,.F.);
#94490=ADVANCED_FACE('',(#9517),#2886,.F.);
#94491=ADVANCED_FACE('',(#9518),#90930,.F.);
#94492=ADVANCED_FACE('',(#9519),#90931,.F.);
#94493=ADVANCED_FACE('',(#9520),#2887,.F.);
#94494=ADVANCED_FACE('',(#9521),#2888,.F.);
#94495=ADVANCED_FACE('',(#9522),#90932,.F.);
#94496=ADVANCED_FACE('',(#9523),#90933,.F.);
#94497=ADVANCED_FACE('',(#9524),#2889,.F.);
#94498=ADVANCED_FACE('',(#9525),#90934,.F.);
#94499=ADVANCED_FACE('',(#9526),#90935,.F.);
#94500=ADVANCED_FACE('',(#9527),#2890,.F.);
#94501=ADVANCED_FACE('',(#9528),#90936,.F.);
#94502=ADVANCED_FACE('',(#9529),#90937,.F.);
#94503=ADVANCED_FACE('',(#9530),#2891,.F.);
#94504=ADVANCED_FACE('',(#9531),#2892,.F.);
#94505=ADVANCED_FACE('',(#9532),#90938,.F.);
#94506=ADVANCED_FACE('',(#9533),#90939,.F.);
#94507=ADVANCED_FACE('',(#9534),#2893,.F.);
#94508=ADVANCED_FACE('',(#9535),#90940,.F.);
#94509=ADVANCED_FACE('',(#9536),#5852,.F.);
#94510=ADVANCED_FACE('',(#9537),#2894,.F.);
#94511=ADVANCED_FACE('',(#9538),#2895,.F.);
#94512=ADVANCED_FACE('',(#9539),#90941,.F.);
#94513=ADVANCED_FACE('',(#9540),#90942,.F.);
#94514=ADVANCED_FACE('',(#9541),#2896,.F.);
#94515=ADVANCED_FACE('',(#9542),#2897,.F.);
#94516=ADVANCED_FACE('',(#9543),#5853,.F.);
#94517=ADVANCED_FACE('',(#9544),#90943,.F.);
#94518=ADVANCED_FACE('',(#9545),#2898,.F.);
#94519=ADVANCED_FACE('',(#9546),#90944,.F.);
#94520=ADVANCED_FACE('',(#9547),#90945,.F.);
#94521=ADVANCED_FACE('',(#9548),#2899,.F.);
#94522=ADVANCED_FACE('',(#9549),#2900,.F.);
#94523=ADVANCED_FACE('',(#9550),#90946,.F.);
#94524=ADVANCED_FACE('',(#9551),#90947,.F.);
#94525=ADVANCED_FACE('',(#9552),#2901,.F.);
#94526=ADVANCED_FACE('',(#9553),#90948,.F.);
#94527=ADVANCED_FACE('',(#9554),#90949,.F.);
#94528=ADVANCED_FACE('',(#9555),#2902,.F.);
#94529=ADVANCED_FACE('',(#9556),#90950,.F.);
#94530=ADVANCED_FACE('',(#9557),#90951,.F.);
#94531=ADVANCED_FACE('',(#9558),#2903,.F.);
#94532=ADVANCED_FACE('',(#9559),#2904,.F.);
#94533=ADVANCED_FACE('',(#9560),#90952,.F.);
#94534=ADVANCED_FACE('',(#9561),#90953,.F.);
#94535=ADVANCED_FACE('',(#9562),#2905,.F.);
#94536=ADVANCED_FACE('',(#9563),#90954,.F.);
#94537=ADVANCED_FACE('',(#9564),#5854,.F.);
#94538=ADVANCED_FACE('',(#9565),#2906,.F.);
#94539=ADVANCED_FACE('',(#9566),#2907,.F.);
#94540=ADVANCED_FACE('',(#9567),#90955,.F.);
#94541=ADVANCED_FACE('',(#9568),#90956,.F.);
#94542=ADVANCED_FACE('',(#9569),#2908,.F.);
#94543=ADVANCED_FACE('',(#9570),#2909,.F.);
#94544=ADVANCED_FACE('',(#9571),#5855,.F.);
#94545=ADVANCED_FACE('',(#9572),#90957,.F.);
#94546=ADVANCED_FACE('',(#9573),#2910,.F.);
#94547=ADVANCED_FACE('',(#9574),#90958,.F.);
#94548=ADVANCED_FACE('',(#9575),#90959,.F.);
#94549=ADVANCED_FACE('',(#9576),#2911,.F.);
#94550=ADVANCED_FACE('',(#9577),#2912,.F.);
#94551=ADVANCED_FACE('',(#9578),#90960,.F.);
#94552=ADVANCED_FACE('',(#9579),#90961,.F.);
#94553=ADVANCED_FACE('',(#9580),#2913,.F.);
#94554=ADVANCED_FACE('',(#9581),#90962,.F.);
#94555=ADVANCED_FACE('',(#9582),#90963,.F.);
#94556=ADVANCED_FACE('',(#9583),#2914,.F.);
#94557=ADVANCED_FACE('',(#9584),#90964,.F.);
#94558=ADVANCED_FACE('',(#9585),#90965,.F.);
#94559=ADVANCED_FACE('',(#9586),#2915,.F.);
#94560=ADVANCED_FACE('',(#9587),#2916,.F.);
#94561=ADVANCED_FACE('',(#9588),#90966,.F.);
#94562=ADVANCED_FACE('',(#9589),#90967,.F.);
#94563=ADVANCED_FACE('',(#9590),#2917,.F.);
#94564=ADVANCED_FACE('',(#9591),#90968,.F.);
#94565=ADVANCED_FACE('',(#9592),#5856,.F.);
#94566=ADVANCED_FACE('',(#9593),#2918,.F.);
#94567=ADVANCED_FACE('',(#9594),#2919,.F.);
#94568=ADVANCED_FACE('',(#9595),#90969,.F.);
#94569=ADVANCED_FACE('',(#9596),#90970,.F.);
#94570=ADVANCED_FACE('',(#9597),#2920,.F.);
#94571=ADVANCED_FACE('',(#9598),#2921,.F.);
#94572=ADVANCED_FACE('',(#9599),#5857,.F.);
#94573=ADVANCED_FACE('',(#9600),#90971,.F.);
#94574=ADVANCED_FACE('',(#9601),#2922,.F.);
#94575=ADVANCED_FACE('',(#9602),#90972,.F.);
#94576=ADVANCED_FACE('',(#9603),#90973,.F.);
#94577=ADVANCED_FACE('',(#9604),#2923,.F.);
#94578=ADVANCED_FACE('',(#9605),#2924,.F.);
#94579=ADVANCED_FACE('',(#9606),#90974,.F.);
#94580=ADVANCED_FACE('',(#9607),#90975,.F.);
#94581=ADVANCED_FACE('',(#9608),#2925,.F.);
#94582=ADVANCED_FACE('',(#9609),#90976,.F.);
#94583=ADVANCED_FACE('',(#9610),#90977,.F.);
#94584=ADVANCED_FACE('',(#9611),#2926,.F.);
#94585=ADVANCED_FACE('',(#9612),#90978,.F.);
#94586=ADVANCED_FACE('',(#9613),#90979,.F.);
#94587=ADVANCED_FACE('',(#9614),#2927,.F.);
#94588=ADVANCED_FACE('',(#9615),#2928,.F.);
#94589=ADVANCED_FACE('',(#9616),#90980,.F.);
#94590=ADVANCED_FACE('',(#9617),#90981,.F.);
#94591=ADVANCED_FACE('',(#9618),#2929,.F.);
#94592=ADVANCED_FACE('',(#9619),#90982,.F.);
#94593=ADVANCED_FACE('',(#9620),#5858,.F.);
#94594=ADVANCED_FACE('',(#9621),#2930,.F.);
#94595=ADVANCED_FACE('',(#9622),#2931,.F.);
#94596=ADVANCED_FACE('',(#9623),#90983,.F.);
#94597=ADVANCED_FACE('',(#9624),#90984,.F.);
#94598=ADVANCED_FACE('',(#9625),#2932,.F.);
#94599=ADVANCED_FACE('',(#9626),#2933,.F.);
#94600=ADVANCED_FACE('',(#9627),#5859,.F.);
#94601=ADVANCED_FACE('',(#9628),#90985,.F.);
#94602=ADVANCED_FACE('',(#9629),#2934,.F.);
#94603=ADVANCED_FACE('',(#9630),#90986,.F.);
#94604=ADVANCED_FACE('',(#9631),#90987,.F.);
#94605=ADVANCED_FACE('',(#9632),#2935,.F.);
#94606=ADVANCED_FACE('',(#9633),#2936,.F.);
#94607=ADVANCED_FACE('',(#9634),#90988,.F.);
#94608=ADVANCED_FACE('',(#9635),#90989,.F.);
#94609=ADVANCED_FACE('',(#9636),#2937,.F.);
#94610=ADVANCED_FACE('',(#9637),#90990,.F.);
#94611=ADVANCED_FACE('',(#9638),#90991,.F.);
#94612=ADVANCED_FACE('',(#9639),#2938,.F.);
#94613=ADVANCED_FACE('',(#9640),#90992,.F.);
#94614=ADVANCED_FACE('',(#9641),#90993,.F.);
#94615=ADVANCED_FACE('',(#9642),#2939,.F.);
#94616=ADVANCED_FACE('',(#9643),#2940,.F.);
#94617=ADVANCED_FACE('',(#9644),#90994,.F.);
#94618=ADVANCED_FACE('',(#9645),#90995,.F.);
#94619=ADVANCED_FACE('',(#9646),#2941,.F.);
#94620=ADVANCED_FACE('',(#9647),#90996,.F.);
#94621=ADVANCED_FACE('',(#9648),#5860,.F.);
#94622=ADVANCED_FACE('',(#9649),#2942,.F.);
#94623=ADVANCED_FACE('',(#9650),#2943,.F.);
#94624=ADVANCED_FACE('',(#9651),#90997,.F.);
#94625=ADVANCED_FACE('',(#9652),#90998,.F.);
#94626=ADVANCED_FACE('',(#9653),#2944,.F.);
#94627=ADVANCED_FACE('',(#9654),#2945,.F.);
#94628=ADVANCED_FACE('',(#9655),#5861,.F.);
#94629=ADVANCED_FACE('',(#9656),#90999,.F.);
#94630=ADVANCED_FACE('',(#9657),#2946,.F.);
#94631=ADVANCED_FACE('',(#9658),#91000,.F.);
#94632=ADVANCED_FACE('',(#9659),#91001,.F.);
#94633=ADVANCED_FACE('',(#9660),#2947,.F.);
#94634=ADVANCED_FACE('',(#9661),#2948,.F.);
#94635=ADVANCED_FACE('',(#9662),#91002,.F.);
#94636=ADVANCED_FACE('',(#9663),#91003,.F.);
#94637=ADVANCED_FACE('',(#9664),#2949,.F.);
#94638=ADVANCED_FACE('',(#9665),#91004,.F.);
#94639=ADVANCED_FACE('',(#9666),#91005,.F.);
#94640=ADVANCED_FACE('',(#9667),#2950,.F.);
#94641=ADVANCED_FACE('',(#9668),#91006,.F.);
#94642=ADVANCED_FACE('',(#9669),#91007,.F.);
#94643=ADVANCED_FACE('',(#9670),#2951,.F.);
#94644=ADVANCED_FACE('',(#9671),#2952,.F.);
#94645=ADVANCED_FACE('',(#9672),#91008,.F.);
#94646=ADVANCED_FACE('',(#9673),#91009,.F.);
#94647=ADVANCED_FACE('',(#9674),#2953,.F.);
#94648=ADVANCED_FACE('',(#9675),#91010,.F.);
#94649=ADVANCED_FACE('',(#9676),#5862,.F.);
#94650=ADVANCED_FACE('',(#9677),#2954,.F.);
#94651=ADVANCED_FACE('',(#9678),#2955,.F.);
#94652=ADVANCED_FACE('',(#9679),#91011,.F.);
#94653=ADVANCED_FACE('',(#9680),#91012,.F.);
#94654=ADVANCED_FACE('',(#9681),#2956,.F.);
#94655=ADVANCED_FACE('',(#9682),#2957,.F.);
#94656=ADVANCED_FACE('',(#9683),#5863,.F.);
#94657=ADVANCED_FACE('',(#9684),#91013,.F.);
#94658=ADVANCED_FACE('',(#9685),#2958,.F.);
#94659=ADVANCED_FACE('',(#9686),#91014,.F.);
#94660=ADVANCED_FACE('',(#9687),#91015,.F.);
#94661=ADVANCED_FACE('',(#9688),#2959,.F.);
#94662=ADVANCED_FACE('',(#9689),#2960,.F.);
#94663=ADVANCED_FACE('',(#9690),#91016,.F.);
#94664=ADVANCED_FACE('',(#9691),#91017,.F.);
#94665=ADVANCED_FACE('',(#9692),#2961,.F.);
#94666=ADVANCED_FACE('',(#9693),#91018,.F.);
#94667=ADVANCED_FACE('',(#9694),#91019,.F.);
#94668=ADVANCED_FACE('',(#9695),#2962,.F.);
#94669=ADVANCED_FACE('',(#9696),#91020,.F.);
#94670=ADVANCED_FACE('',(#9697),#91021,.F.);
#94671=ADVANCED_FACE('',(#9698),#2963,.F.);
#94672=ADVANCED_FACE('',(#9699),#2964,.F.);
#94673=ADVANCED_FACE('',(#9700),#91022,.F.);
#94674=ADVANCED_FACE('',(#9701),#91023,.F.);
#94675=ADVANCED_FACE('',(#9702),#2965,.F.);
#94676=ADVANCED_FACE('',(#9703),#91024,.F.);
#94677=ADVANCED_FACE('',(#9704),#5864,.F.);
#94678=ADVANCED_FACE('',(#9705),#2966,.F.);
#94679=ADVANCED_FACE('',(#9706),#2967,.F.);
#94680=ADVANCED_FACE('',(#9707),#91025,.F.);
#94681=ADVANCED_FACE('',(#9708),#91026,.F.);
#94682=ADVANCED_FACE('',(#9709),#2968,.F.);
#94683=ADVANCED_FACE('',(#9710),#2969,.F.);
#94684=ADVANCED_FACE('',(#9711),#5865,.F.);
#94685=ADVANCED_FACE('',(#9712),#91027,.F.);
#94686=ADVANCED_FACE('',(#9713),#2970,.F.);
#94687=ADVANCED_FACE('',(#9714),#91028,.F.);
#94688=ADVANCED_FACE('',(#9715),#91029,.F.);
#94689=ADVANCED_FACE('',(#9716),#2971,.F.);
#94690=ADVANCED_FACE('',(#9717),#2972,.F.);
#94691=ADVANCED_FACE('',(#9718),#91030,.F.);
#94692=ADVANCED_FACE('',(#9719),#91031,.F.);
#94693=ADVANCED_FACE('',(#9720),#2973,.F.);
#94694=ADVANCED_FACE('',(#9721),#91032,.F.);
#94695=ADVANCED_FACE('',(#9722),#91033,.F.);
#94696=ADVANCED_FACE('',(#9723),#2974,.F.);
#94697=ADVANCED_FACE('',(#9724),#91034,.F.);
#94698=ADVANCED_FACE('',(#9725),#91035,.F.);
#94699=ADVANCED_FACE('',(#9726),#2975,.F.);
#94700=ADVANCED_FACE('',(#9727),#2976,.F.);
#94701=ADVANCED_FACE('',(#9728),#91036,.F.);
#94702=ADVANCED_FACE('',(#9729),#91037,.F.);
#94703=ADVANCED_FACE('',(#9730),#2977,.F.);
#94704=ADVANCED_FACE('',(#9731),#91038,.F.);
#94705=ADVANCED_FACE('',(#9732),#5866,.F.);
#94706=ADVANCED_FACE('',(#9733),#2978,.F.);
#94707=ADVANCED_FACE('',(#9734),#2979,.F.);
#94708=ADVANCED_FACE('',(#9735),#91039,.F.);
#94709=ADVANCED_FACE('',(#9736),#91040,.F.);
#94710=ADVANCED_FACE('',(#9737),#2980,.F.);
#94711=ADVANCED_FACE('',(#9738),#2981,.F.);
#94712=ADVANCED_FACE('',(#9739),#5867,.F.);
#94713=ADVANCED_FACE('',(#9740),#91041,.F.);
#94714=ADVANCED_FACE('',(#9741),#2982,.F.);
#94715=ADVANCED_FACE('',(#9742),#91042,.F.);
#94716=ADVANCED_FACE('',(#9743),#91043,.F.);
#94717=ADVANCED_FACE('',(#9744),#2983,.F.);
#94718=ADVANCED_FACE('',(#9745),#2984,.F.);
#94719=ADVANCED_FACE('',(#9746),#91044,.F.);
#94720=ADVANCED_FACE('',(#9747),#91045,.F.);
#94721=ADVANCED_FACE('',(#9748),#2985,.F.);
#94722=ADVANCED_FACE('',(#9749),#91046,.F.);
#94723=ADVANCED_FACE('',(#9750),#91047,.F.);
#94724=ADVANCED_FACE('',(#9751),#2986,.F.);
#94725=ADVANCED_FACE('',(#9752),#91048,.F.);
#94726=ADVANCED_FACE('',(#9753),#91049,.F.);
#94727=ADVANCED_FACE('',(#9754),#2987,.F.);
#94728=ADVANCED_FACE('',(#9755),#2988,.F.);
#94729=ADVANCED_FACE('',(#9756),#91050,.F.);
#94730=ADVANCED_FACE('',(#9757),#91051,.F.);
#94731=ADVANCED_FACE('',(#9758),#2989,.F.);
#94732=ADVANCED_FACE('',(#9759),#91052,.F.);
#94733=ADVANCED_FACE('',(#9760),#5868,.F.);
#94734=ADVANCED_FACE('',(#9761),#2990,.F.);
#94735=ADVANCED_FACE('',(#9762),#2991,.F.);
#94736=ADVANCED_FACE('',(#9763),#91053,.F.);
#94737=ADVANCED_FACE('',(#9764),#91054,.F.);
#94738=ADVANCED_FACE('',(#9765),#2992,.F.);
#94739=ADVANCED_FACE('',(#9766),#2993,.F.);
#94740=ADVANCED_FACE('',(#9767),#5869,.F.);
#94741=ADVANCED_FACE('',(#9768),#91055,.F.);
#94742=ADVANCED_FACE('',(#9769),#2994,.F.);
#94743=ADVANCED_FACE('',(#9770),#91056,.F.);
#94744=ADVANCED_FACE('',(#9771),#91057,.F.);
#94745=ADVANCED_FACE('',(#9772),#2995,.F.);
#94746=ADVANCED_FACE('',(#9773),#2996,.F.);
#94747=ADVANCED_FACE('',(#9774),#91058,.F.);
#94748=ADVANCED_FACE('',(#9775),#91059,.F.);
#94749=ADVANCED_FACE('',(#9776),#2997,.F.);
#94750=ADVANCED_FACE('',(#9777),#91060,.F.);
#94751=ADVANCED_FACE('',(#9778),#91061,.F.);
#94752=ADVANCED_FACE('',(#9779),#2998,.F.);
#94753=ADVANCED_FACE('',(#9780),#91062,.F.);
#94754=ADVANCED_FACE('',(#9781),#91063,.F.);
#94755=ADVANCED_FACE('',(#9782),#2999,.F.);
#94756=ADVANCED_FACE('',(#9783),#3000,.F.);
#94757=ADVANCED_FACE('',(#9784),#91064,.F.);
#94758=ADVANCED_FACE('',(#9785),#91065,.F.);
#94759=ADVANCED_FACE('',(#9786),#3001,.F.);
#94760=ADVANCED_FACE('',(#9787),#91066,.F.);
#94761=ADVANCED_FACE('',(#9788),#5870,.F.);
#94762=ADVANCED_FACE('',(#9789),#3002,.F.);
#94763=ADVANCED_FACE('',(#9790),#3003,.F.);
#94764=ADVANCED_FACE('',(#9791),#91067,.F.);
#94765=ADVANCED_FACE('',(#9792),#91068,.F.);
#94766=ADVANCED_FACE('',(#9793),#3004,.F.);
#94767=ADVANCED_FACE('',(#9794),#3005,.F.);
#94768=ADVANCED_FACE('',(#9795),#5871,.F.);
#94769=ADVANCED_FACE('',(#9796),#91069,.F.);
#94770=ADVANCED_FACE('',(#9797),#3006,.F.);
#94771=ADVANCED_FACE('',(#9798),#91070,.F.);
#94772=ADVANCED_FACE('',(#9799),#91071,.F.);
#94773=ADVANCED_FACE('',(#9800),#3007,.F.);
#94774=ADVANCED_FACE('',(#9801),#3008,.F.);
#94775=ADVANCED_FACE('',(#9802),#91072,.F.);
#94776=ADVANCED_FACE('',(#9803),#91073,.F.);
#94777=ADVANCED_FACE('',(#9804),#3009,.F.);
#94778=ADVANCED_FACE('',(#9805),#91074,.F.);
#94779=ADVANCED_FACE('',(#9806),#91075,.F.);
#94780=ADVANCED_FACE('',(#9807),#3010,.F.);
#94781=ADVANCED_FACE('',(#9808),#91076,.F.);
#94782=ADVANCED_FACE('',(#9809),#91077,.F.);
#94783=ADVANCED_FACE('',(#9810),#3011,.F.);
#94784=ADVANCED_FACE('',(#9811),#3012,.F.);
#94785=ADVANCED_FACE('',(#9812),#91078,.F.);
#94786=ADVANCED_FACE('',(#9813),#91079,.F.);
#94787=ADVANCED_FACE('',(#9814),#3013,.F.);
#94788=ADVANCED_FACE('',(#9815),#91080,.F.);
#94789=ADVANCED_FACE('',(#9816),#5872,.F.);
#94790=ADVANCED_FACE('',(#9817),#3014,.F.);
#94791=ADVANCED_FACE('',(#9818),#3015,.F.);
#94792=ADVANCED_FACE('',(#9819),#91081,.F.);
#94793=ADVANCED_FACE('',(#9820),#91082,.F.);
#94794=ADVANCED_FACE('',(#9821),#3016,.F.);
#94795=ADVANCED_FACE('',(#9822),#3017,.F.);
#94796=ADVANCED_FACE('',(#9823),#5873,.F.);
#94797=ADVANCED_FACE('',(#9824),#91083,.F.);
#94798=ADVANCED_FACE('',(#9825),#3018,.F.);
#94799=ADVANCED_FACE('',(#9826),#91084,.F.);
#94800=ADVANCED_FACE('',(#9827),#91085,.F.);
#94801=ADVANCED_FACE('',(#9828),#3019,.F.);
#94802=ADVANCED_FACE('',(#9829),#3020,.F.);
#94803=ADVANCED_FACE('',(#9830),#91086,.F.);
#94804=ADVANCED_FACE('',(#9831),#91087,.F.);
#94805=ADVANCED_FACE('',(#9832),#3021,.F.);
#94806=ADVANCED_FACE('',(#9833),#91088,.F.);
#94807=ADVANCED_FACE('',(#9834),#91089,.F.);
#94808=ADVANCED_FACE('',(#9835),#3022,.F.);
#94809=ADVANCED_FACE('',(#9836),#91090,.F.);
#94810=ADVANCED_FACE('',(#9837),#91091,.F.);
#94811=ADVANCED_FACE('',(#9838),#3023,.F.);
#94812=ADVANCED_FACE('',(#9839),#3024,.F.);
#94813=ADVANCED_FACE('',(#9840),#91092,.F.);
#94814=ADVANCED_FACE('',(#9841),#91093,.F.);
#94815=ADVANCED_FACE('',(#9842),#3025,.F.);
#94816=ADVANCED_FACE('',(#9843),#91094,.F.);
#94817=ADVANCED_FACE('',(#9844),#5874,.F.);
#94818=ADVANCED_FACE('',(#9845),#3026,.F.);
#94819=ADVANCED_FACE('',(#9846),#3027,.F.);
#94820=ADVANCED_FACE('',(#9847),#91095,.F.);
#94821=ADVANCED_FACE('',(#9848),#91096,.F.);
#94822=ADVANCED_FACE('',(#9849),#3028,.F.);
#94823=ADVANCED_FACE('',(#9850),#3029,.F.);
#94824=ADVANCED_FACE('',(#9851),#5875,.F.);
#94825=ADVANCED_FACE('',(#9852),#91097,.F.);
#94826=ADVANCED_FACE('',(#9853),#3030,.F.);
#94827=ADVANCED_FACE('',(#9854),#91098,.F.);
#94828=ADVANCED_FACE('',(#9855),#91099,.F.);
#94829=ADVANCED_FACE('',(#9856),#3031,.F.);
#94830=ADVANCED_FACE('',(#9857),#3032,.F.);
#94831=ADVANCED_FACE('',(#9858),#91100,.F.);
#94832=ADVANCED_FACE('',(#9859),#91101,.F.);
#94833=ADVANCED_FACE('',(#9860),#3033,.F.);
#94834=ADVANCED_FACE('',(#9861),#91102,.F.);
#94835=ADVANCED_FACE('',(#9862),#91103,.F.);
#94836=ADVANCED_FACE('',(#9863),#3034,.F.);
#94837=ADVANCED_FACE('',(#9864),#91104,.F.);
#94838=ADVANCED_FACE('',(#9865),#91105,.F.);
#94839=ADVANCED_FACE('',(#9866),#3035,.F.);
#94840=ADVANCED_FACE('',(#9867),#3036,.F.);
#94841=ADVANCED_FACE('',(#9868),#91106,.F.);
#94842=ADVANCED_FACE('',(#9869),#91107,.F.);
#94843=ADVANCED_FACE('',(#9870),#3037,.F.);
#94844=ADVANCED_FACE('',(#9871),#91108,.F.);
#94845=ADVANCED_FACE('',(#9872),#5876,.F.);
#94846=ADVANCED_FACE('',(#9873),#3038,.F.);
#94847=ADVANCED_FACE('',(#9874),#3039,.F.);
#94848=ADVANCED_FACE('',(#9875),#91109,.F.);
#94849=ADVANCED_FACE('',(#9876),#91110,.F.);
#94850=ADVANCED_FACE('',(#9877),#3040,.F.);
#94851=ADVANCED_FACE('',(#9878),#3041,.F.);
#94852=ADVANCED_FACE('',(#9879),#5877,.F.);
#94853=ADVANCED_FACE('',(#9880),#91111,.F.);
#94854=ADVANCED_FACE('',(#9881),#3042,.F.);
#94855=ADVANCED_FACE('',(#9882),#91112,.F.);
#94856=ADVANCED_FACE('',(#9883),#91113,.F.);
#94857=ADVANCED_FACE('',(#9884),#3043,.F.);
#94858=ADVANCED_FACE('',(#9885),#3044,.F.);
#94859=ADVANCED_FACE('',(#9886),#91114,.F.);
#94860=ADVANCED_FACE('',(#9887),#91115,.F.);
#94861=ADVANCED_FACE('',(#9888),#3045,.F.);
#94862=ADVANCED_FACE('',(#9889),#91116,.F.);
#94863=ADVANCED_FACE('',(#9890),#91117,.F.);
#94864=ADVANCED_FACE('',(#9891),#3046,.F.);
#94865=ADVANCED_FACE('',(#9892),#91118,.F.);
#94866=ADVANCED_FACE('',(#9893),#91119,.F.);
#94867=ADVANCED_FACE('',(#9894),#3047,.F.);
#94868=ADVANCED_FACE('',(#9895),#3048,.F.);
#94869=ADVANCED_FACE('',(#9896),#91120,.F.);
#94870=ADVANCED_FACE('',(#9897),#91121,.F.);
#94871=ADVANCED_FACE('',(#9898),#3049,.F.);
#94872=ADVANCED_FACE('',(#9899),#91122,.F.);
#94873=ADVANCED_FACE('',(#9900),#3050,.F.);
#94874=ADVANCED_FACE('',(#9901),#3051,.F.);
#94875=ADVANCED_FACE('',(#9902),#91123,.F.);
#94876=ADVANCED_FACE('',(#9903),#91124,.F.);
#94877=ADVANCED_FACE('',(#9904),#3052,.F.);
#94878=ADVANCED_FACE('',(#9905),#3053,.F.);
#94879=ADVANCED_FACE('',(#9906),#91125,.F.);
#94880=ADVANCED_FACE('',(#9907),#3054,.F.);
#94881=ADVANCED_FACE('',(#9908),#91126,.F.);
#94882=ADVANCED_FACE('',(#9909),#91127,.F.);
#94883=ADVANCED_FACE('',(#9910),#3055,.F.);
#94884=ADVANCED_FACE('',(#9911),#3056,.F.);
#94885=ADVANCED_FACE('',(#9912),#91128,.F.);
#94886=ADVANCED_FACE('',(#9913),#91129,.F.);
#94887=ADVANCED_FACE('',(#9914),#3057,.F.);
#94888=ADVANCED_FACE('',(#9915),#91130,.F.);
#94889=ADVANCED_FACE('',(#9916),#91131,.F.);
#94890=ADVANCED_FACE('',(#9917),#3058,.F.);
#94891=ADVANCED_FACE('',(#9918),#91132,.F.);
#94892=ADVANCED_FACE('',(#9919),#91133,.F.);
#94893=ADVANCED_FACE('',(#9920),#3059,.F.);
#94894=ADVANCED_FACE('',(#9921),#3060,.F.);
#94895=ADVANCED_FACE('',(#9922),#91134,.F.);
#94896=ADVANCED_FACE('',(#9923),#91135,.F.);
#94897=ADVANCED_FACE('',(#9924),#3061,.F.);
#94898=ADVANCED_FACE('',(#9925),#91136,.F.);
#94899=ADVANCED_FACE('',(#9926),#5878,.F.);
#94900=ADVANCED_FACE('',(#9927),#3062,.F.);
#94901=ADVANCED_FACE('',(#9928),#3063,.F.);
#94902=ADVANCED_FACE('',(#9929),#91137,.F.);
#94903=ADVANCED_FACE('',(#9930),#91138,.F.);
#94904=ADVANCED_FACE('',(#9931),#3064,.F.);
#94905=ADVANCED_FACE('',(#9932),#3065,.F.);
#94906=ADVANCED_FACE('',(#9933),#5879,.F.);
#94907=ADVANCED_FACE('',(#9934),#91139,.F.);
#94908=ADVANCED_FACE('',(#9935),#3066,.F.);
#94909=ADVANCED_FACE('',(#9936),#91140,.F.);
#94910=ADVANCED_FACE('',(#9937),#91141,.F.);
#94911=ADVANCED_FACE('',(#9938),#3067,.F.);
#94912=ADVANCED_FACE('',(#9939),#3068,.F.);
#94913=ADVANCED_FACE('',(#9940),#91142,.F.);
#94914=ADVANCED_FACE('',(#9941),#91143,.F.);
#94915=ADVANCED_FACE('',(#9942),#3069,.F.);
#94916=ADVANCED_FACE('',(#9943),#91144,.F.);
#94917=ADVANCED_FACE('',(#9944),#91145,.F.);
#94918=ADVANCED_FACE('',(#9945),#3070,.F.);
#94919=ADVANCED_FACE('',(#9946),#91146,.F.);
#94920=ADVANCED_FACE('',(#9947),#91147,.F.);
#94921=ADVANCED_FACE('',(#9948),#3071,.F.);
#94922=ADVANCED_FACE('',(#9949),#3072,.F.);
#94923=ADVANCED_FACE('',(#9950),#91148,.F.);
#94924=ADVANCED_FACE('',(#9951),#91149,.F.);
#94925=ADVANCED_FACE('',(#9952),#3073,.F.);
#94926=ADVANCED_FACE('',(#9953),#91150,.F.);
#94927=ADVANCED_FACE('',(#9954),#5880,.F.);
#94928=ADVANCED_FACE('',(#9955),#3074,.F.);
#94929=ADVANCED_FACE('',(#9956),#3075,.F.);
#94930=ADVANCED_FACE('',(#9957),#91151,.F.);
#94931=ADVANCED_FACE('',(#9958),#91152,.F.);
#94932=ADVANCED_FACE('',(#9959),#3076,.F.);
#94933=ADVANCED_FACE('',(#9960),#3077,.F.);
#94934=ADVANCED_FACE('',(#9961),#5881,.F.);
#94935=ADVANCED_FACE('',(#9962),#91153,.F.);
#94936=ADVANCED_FACE('',(#9963),#3078,.F.);
#94937=ADVANCED_FACE('',(#9964),#91154,.F.);
#94938=ADVANCED_FACE('',(#9965),#91155,.F.);
#94939=ADVANCED_FACE('',(#9966),#3079,.F.);
#94940=ADVANCED_FACE('',(#9967),#3080,.F.);
#94941=ADVANCED_FACE('',(#9968),#91156,.F.);
#94942=ADVANCED_FACE('',(#9969),#91157,.F.);
#94943=ADVANCED_FACE('',(#9970),#3081,.F.);
#94944=ADVANCED_FACE('',(#9971),#91158,.F.);
#94945=ADVANCED_FACE('',(#9972),#91159,.F.);
#94946=ADVANCED_FACE('',(#9973),#3082,.F.);
#94947=ADVANCED_FACE('',(#9974),#91160,.F.);
#94948=ADVANCED_FACE('',(#9975),#91161,.F.);
#94949=ADVANCED_FACE('',(#9976),#3083,.F.);
#94950=ADVANCED_FACE('',(#9977),#3084,.F.);
#94951=ADVANCED_FACE('',(#9978),#91162,.F.);
#94952=ADVANCED_FACE('',(#9979),#91163,.F.);
#94953=ADVANCED_FACE('',(#9980),#3085,.F.);
#94954=ADVANCED_FACE('',(#9981),#91164,.F.);
#94955=ADVANCED_FACE('',(#9982),#5882,.F.);
#94956=ADVANCED_FACE('',(#9983),#3086,.F.);
#94957=ADVANCED_FACE('',(#9984),#3087,.F.);
#94958=ADVANCED_FACE('',(#9985),#91165,.F.);
#94959=ADVANCED_FACE('',(#9986),#91166,.F.);
#94960=ADVANCED_FACE('',(#9987),#3088,.F.);
#94961=ADVANCED_FACE('',(#9988),#3089,.F.);
#94962=ADVANCED_FACE('',(#9989),#5883,.F.);
#94963=ADVANCED_FACE('',(#9990),#91167,.F.);
#94964=ADVANCED_FACE('',(#9991),#3090,.F.);
#94965=ADVANCED_FACE('',(#9992),#91168,.F.);
#94966=ADVANCED_FACE('',(#9993),#91169,.F.);
#94967=ADVANCED_FACE('',(#9994),#3091,.F.);
#94968=ADVANCED_FACE('',(#9995),#3092,.F.);
#94969=ADVANCED_FACE('',(#9996),#91170,.F.);
#94970=ADVANCED_FACE('',(#9997),#91171,.F.);
#94971=ADVANCED_FACE('',(#9998),#3093,.F.);
#94972=ADVANCED_FACE('',(#9999),#91172,.F.);
#94973=ADVANCED_FACE('',(#10000),#91173,.F.);
#94974=ADVANCED_FACE('',(#10001),#3094,.F.);
#94975=ADVANCED_FACE('',(#10002),#91174,.F.);
#94976=ADVANCED_FACE('',(#10003),#91175,.F.);
#94977=ADVANCED_FACE('',(#10004),#3095,.F.);
#94978=ADVANCED_FACE('',(#10005),#3096,.F.);
#94979=ADVANCED_FACE('',(#10006),#91176,.F.);
#94980=ADVANCED_FACE('',(#10007),#91177,.F.);
#94981=ADVANCED_FACE('',(#10008),#3097,.F.);
#94982=ADVANCED_FACE('',(#10009),#91178,.F.);
#94983=ADVANCED_FACE('',(#10010),#5884,.F.);
#94984=ADVANCED_FACE('',(#10011),#3098,.F.);
#94985=ADVANCED_FACE('',(#10012),#3099,.F.);
#94986=ADVANCED_FACE('',(#10013),#91179,.F.);
#94987=ADVANCED_FACE('',(#10014),#91180,.F.);
#94988=ADVANCED_FACE('',(#10015),#3100,.F.);
#94989=ADVANCED_FACE('',(#10016),#3101,.F.);
#94990=ADVANCED_FACE('',(#10017),#5885,.F.);
#94991=ADVANCED_FACE('',(#10018),#91181,.F.);
#94992=ADVANCED_FACE('',(#10019),#3102,.F.);
#94993=ADVANCED_FACE('',(#10020),#91182,.F.);
#94994=ADVANCED_FACE('',(#10021),#91183,.F.);
#94995=ADVANCED_FACE('',(#10022),#3103,.F.);
#94996=ADVANCED_FACE('',(#10023),#3104,.F.);
#94997=ADVANCED_FACE('',(#10024),#91184,.F.);
#94998=ADVANCED_FACE('',(#10025),#91185,.F.);
#94999=ADVANCED_FACE('',(#10026),#3105,.F.);
#95000=ADVANCED_FACE('',(#10027),#91186,.F.);
#95001=ADVANCED_FACE('',(#10028),#91187,.F.);
#95002=ADVANCED_FACE('',(#10029),#3106,.F.);
#95003=ADVANCED_FACE('',(#10030),#91188,.F.);
#95004=ADVANCED_FACE('',(#10031),#91189,.F.);
#95005=ADVANCED_FACE('',(#10032),#3107,.F.);
#95006=ADVANCED_FACE('',(#10033),#3108,.F.);
#95007=ADVANCED_FACE('',(#10034),#91190,.F.);
#95008=ADVANCED_FACE('',(#10035),#91191,.F.);
#95009=ADVANCED_FACE('',(#10036),#3109,.F.);
#95010=ADVANCED_FACE('',(#10037),#91192,.F.);
#95011=ADVANCED_FACE('',(#10038),#5886,.F.);
#95012=ADVANCED_FACE('',(#10039),#3110,.F.);
#95013=ADVANCED_FACE('',(#10040),#3111,.F.);
#95014=ADVANCED_FACE('',(#10041),#91193,.F.);
#95015=ADVANCED_FACE('',(#10042),#91194,.F.);
#95016=ADVANCED_FACE('',(#10043),#3112,.F.);
#95017=ADVANCED_FACE('',(#10044),#3113,.F.);
#95018=ADVANCED_FACE('',(#10045),#5887,.F.);
#95019=ADVANCED_FACE('',(#10046),#91195,.F.);
#95020=ADVANCED_FACE('',(#10047),#3114,.F.);
#95021=ADVANCED_FACE('',(#10048),#91196,.F.);
#95022=ADVANCED_FACE('',(#10049),#91197,.F.);
#95023=ADVANCED_FACE('',(#10050),#3115,.F.);
#95024=ADVANCED_FACE('',(#10051),#3116,.F.);
#95025=ADVANCED_FACE('',(#10052),#91198,.F.);
#95026=ADVANCED_FACE('',(#10053),#91199,.F.);
#95027=ADVANCED_FACE('',(#10054),#3117,.F.);
#95028=ADVANCED_FACE('',(#10055),#91200,.F.);
#95029=ADVANCED_FACE('',(#10056),#91201,.F.);
#95030=ADVANCED_FACE('',(#10057),#3118,.F.);
#95031=ADVANCED_FACE('',(#10058),#91202,.F.);
#95032=ADVANCED_FACE('',(#10059),#91203,.F.);
#95033=ADVANCED_FACE('',(#10060),#3119,.F.);
#95034=ADVANCED_FACE('',(#10061),#3120,.F.);
#95035=ADVANCED_FACE('',(#10062),#91204,.F.);
#95036=ADVANCED_FACE('',(#10063),#91205,.F.);
#95037=ADVANCED_FACE('',(#10064),#3121,.F.);
#95038=ADVANCED_FACE('',(#10065),#91206,.F.);
#95039=ADVANCED_FACE('',(#10066),#5888,.F.);
#95040=ADVANCED_FACE('',(#10067),#3122,.F.);
#95041=ADVANCED_FACE('',(#10068),#3123,.F.);
#95042=ADVANCED_FACE('',(#10069),#91207,.F.);
#95043=ADVANCED_FACE('',(#10070),#91208,.F.);
#95044=ADVANCED_FACE('',(#10071),#3124,.F.);
#95045=ADVANCED_FACE('',(#10072),#3125,.F.);
#95046=ADVANCED_FACE('',(#10073),#5889,.F.);
#95047=ADVANCED_FACE('',(#10074),#91209,.F.);
#95048=ADVANCED_FACE('',(#10075),#3126,.F.);
#95049=ADVANCED_FACE('',(#10076),#91210,.F.);
#95050=ADVANCED_FACE('',(#10077),#91211,.F.);
#95051=ADVANCED_FACE('',(#10078),#3127,.F.);
#95052=ADVANCED_FACE('',(#10079),#3128,.F.);
#95053=ADVANCED_FACE('',(#10080),#91212,.F.);
#95054=ADVANCED_FACE('',(#10081),#91213,.F.);
#95055=ADVANCED_FACE('',(#10082),#3129,.F.);
#95056=ADVANCED_FACE('',(#10083),#91214,.F.);
#95057=ADVANCED_FACE('',(#10084),#91215,.F.);
#95058=ADVANCED_FACE('',(#10085),#3130,.F.);
#95059=ADVANCED_FACE('',(#10086),#91216,.F.);
#95060=ADVANCED_FACE('',(#10087),#91217,.F.);
#95061=ADVANCED_FACE('',(#10088),#3131,.F.);
#95062=ADVANCED_FACE('',(#10089),#3132,.F.);
#95063=ADVANCED_FACE('',(#10090),#91218,.F.);
#95064=ADVANCED_FACE('',(#10091),#91219,.F.);
#95065=ADVANCED_FACE('',(#10092),#3133,.F.);
#95066=ADVANCED_FACE('',(#10093),#91220,.F.);
#95067=ADVANCED_FACE('',(#10094),#5890,.F.);
#95068=ADVANCED_FACE('',(#10095),#3134,.F.);
#95069=ADVANCED_FACE('',(#10096),#3135,.F.);
#95070=ADVANCED_FACE('',(#10097),#91221,.F.);
#95071=ADVANCED_FACE('',(#10098),#91222,.F.);
#95072=ADVANCED_FACE('',(#10099),#3136,.F.);
#95073=ADVANCED_FACE('',(#10100),#3137,.F.);
#95074=ADVANCED_FACE('',(#10101),#5891,.F.);
#95075=ADVANCED_FACE('',(#10102),#91223,.F.);
#95076=ADVANCED_FACE('',(#10103),#3138,.F.);
#95077=ADVANCED_FACE('',(#10104),#91224,.F.);
#95078=ADVANCED_FACE('',(#10105),#91225,.F.);
#95079=ADVANCED_FACE('',(#10106),#3139,.F.);
#95080=ADVANCED_FACE('',(#10107),#3140,.F.);
#95081=ADVANCED_FACE('',(#10108),#91226,.F.);
#95082=ADVANCED_FACE('',(#10109),#91227,.F.);
#95083=ADVANCED_FACE('',(#10110),#3141,.F.);
#95084=ADVANCED_FACE('',(#10111),#91228,.F.);
#95085=ADVANCED_FACE('',(#10112),#91229,.F.);
#95086=ADVANCED_FACE('',(#10113),#3142,.F.);
#95087=ADVANCED_FACE('',(#10114),#91230,.F.);
#95088=ADVANCED_FACE('',(#10115),#91231,.F.);
#95089=ADVANCED_FACE('',(#10116),#3143,.F.);
#95090=ADVANCED_FACE('',(#10117),#3144,.F.);
#95091=ADVANCED_FACE('',(#10118),#91232,.F.);
#95092=ADVANCED_FACE('',(#10119),#91233,.F.);
#95093=ADVANCED_FACE('',(#10120),#3145,.F.);
#95094=ADVANCED_FACE('',(#10121),#91234,.F.);
#95095=ADVANCED_FACE('',(#10122),#5892,.F.);
#95096=ADVANCED_FACE('',(#10123),#3146,.F.);
#95097=ADVANCED_FACE('',(#10124),#3147,.F.);
#95098=ADVANCED_FACE('',(#10125),#91235,.F.);
#95099=ADVANCED_FACE('',(#10126),#91236,.F.);
#95100=ADVANCED_FACE('',(#10127),#3148,.F.);
#95101=ADVANCED_FACE('',(#10128),#3149,.F.);
#95102=ADVANCED_FACE('',(#10129),#5893,.F.);
#95103=ADVANCED_FACE('',(#10130),#91237,.F.);
#95104=ADVANCED_FACE('',(#10131),#3150,.F.);
#95105=ADVANCED_FACE('',(#10132),#91238,.F.);
#95106=ADVANCED_FACE('',(#10133),#91239,.F.);
#95107=ADVANCED_FACE('',(#10134),#3151,.F.);
#95108=ADVANCED_FACE('',(#10135),#3152,.F.);
#95109=ADVANCED_FACE('',(#10136),#91240,.F.);
#95110=ADVANCED_FACE('',(#10137),#91241,.F.);
#95111=ADVANCED_FACE('',(#10138),#3153,.F.);
#95112=ADVANCED_FACE('',(#10139),#91242,.F.);
#95113=ADVANCED_FACE('',(#10140),#91243,.F.);
#95114=ADVANCED_FACE('',(#10141),#3154,.F.);
#95115=ADVANCED_FACE('',(#10142),#91244,.F.);
#95116=ADVANCED_FACE('',(#10143),#91245,.F.);
#95117=ADVANCED_FACE('',(#10144),#3155,.F.);
#95118=ADVANCED_FACE('',(#10145),#3156,.F.);
#95119=ADVANCED_FACE('',(#10146),#91246,.F.);
#95120=ADVANCED_FACE('',(#10147),#91247,.F.);
#95121=ADVANCED_FACE('',(#10148),#3157,.F.);
#95122=ADVANCED_FACE('',(#10149),#91248,.F.);
#95123=ADVANCED_FACE('',(#10150),#5894,.F.);
#95124=ADVANCED_FACE('',(#10151),#3158,.F.);
#95125=ADVANCED_FACE('',(#10152),#3159,.F.);
#95126=ADVANCED_FACE('',(#10153),#91249,.F.);
#95127=ADVANCED_FACE('',(#10154),#91250,.F.);
#95128=ADVANCED_FACE('',(#10155),#3160,.F.);
#95129=ADVANCED_FACE('',(#10156),#3161,.F.);
#95130=ADVANCED_FACE('',(#10157),#5895,.F.);
#95131=ADVANCED_FACE('',(#10158),#91251,.F.);
#95132=ADVANCED_FACE('',(#10159),#3162,.F.);
#95133=ADVANCED_FACE('',(#10160),#91252,.F.);
#95134=ADVANCED_FACE('',(#10161),#91253,.F.);
#95135=ADVANCED_FACE('',(#10162),#3163,.F.);
#95136=ADVANCED_FACE('',(#10163),#3164,.F.);
#95137=ADVANCED_FACE('',(#10164),#91254,.F.);
#95138=ADVANCED_FACE('',(#10165),#91255,.F.);
#95139=ADVANCED_FACE('',(#10166),#3165,.F.);
#95140=ADVANCED_FACE('',(#10167),#91256,.F.);
#95141=ADVANCED_FACE('',(#10168),#91257,.F.);
#95142=ADVANCED_FACE('',(#10169),#3166,.F.);
#95143=ADVANCED_FACE('',(#10170),#91258,.F.);
#95144=ADVANCED_FACE('',(#10171),#91259,.F.);
#95145=ADVANCED_FACE('',(#10172),#3167,.F.);
#95146=ADVANCED_FACE('',(#10173),#3168,.F.);
#95147=ADVANCED_FACE('',(#10174),#91260,.F.);
#95148=ADVANCED_FACE('',(#10175),#91261,.F.);
#95149=ADVANCED_FACE('',(#10176),#3169,.F.);
#95150=ADVANCED_FACE('',(#10177),#91262,.F.);
#95151=ADVANCED_FACE('',(#10178),#5896,.F.);
#95152=ADVANCED_FACE('',(#10179),#3170,.F.);
#95153=ADVANCED_FACE('',(#10180),#3171,.F.);
#95154=ADVANCED_FACE('',(#10181),#91263,.F.);
#95155=ADVANCED_FACE('',(#10182),#91264,.F.);
#95156=ADVANCED_FACE('',(#10183),#3172,.F.);
#95157=ADVANCED_FACE('',(#10184),#3173,.F.);
#95158=ADVANCED_FACE('',(#10185),#5897,.F.);
#95159=ADVANCED_FACE('',(#10186),#91265,.F.);
#95160=ADVANCED_FACE('',(#10187),#3174,.F.);
#95161=ADVANCED_FACE('',(#10188),#91266,.F.);
#95162=ADVANCED_FACE('',(#10189),#91267,.F.);
#95163=ADVANCED_FACE('',(#10190),#3175,.F.);
#95164=ADVANCED_FACE('',(#10191),#3176,.F.);
#95165=ADVANCED_FACE('',(#10192),#91268,.F.);
#95166=ADVANCED_FACE('',(#10193),#91269,.F.);
#95167=ADVANCED_FACE('',(#10194),#3177,.F.);
#95168=ADVANCED_FACE('',(#10195),#91270,.F.);
#95169=ADVANCED_FACE('',(#10196),#91271,.F.);
#95170=ADVANCED_FACE('',(#10197),#3178,.F.);
#95171=ADVANCED_FACE('',(#10198),#91272,.F.);
#95172=ADVANCED_FACE('',(#10199),#91273,.F.);
#95173=ADVANCED_FACE('',(#10200),#3179,.F.);
#95174=ADVANCED_FACE('',(#10201),#3180,.F.);
#95175=ADVANCED_FACE('',(#10202),#91274,.F.);
#95176=ADVANCED_FACE('',(#10203),#91275,.F.);
#95177=ADVANCED_FACE('',(#10204),#3181,.F.);
#95178=ADVANCED_FACE('',(#10205),#91276,.F.);
#95179=ADVANCED_FACE('',(#10206),#5898,.F.);
#95180=ADVANCED_FACE('',(#10207),#3182,.F.);
#95181=ADVANCED_FACE('',(#10208),#3183,.F.);
#95182=ADVANCED_FACE('',(#10209),#91277,.F.);
#95183=ADVANCED_FACE('',(#10210),#91278,.F.);
#95184=ADVANCED_FACE('',(#10211),#3184,.F.);
#95185=ADVANCED_FACE('',(#10212),#3185,.F.);
#95186=ADVANCED_FACE('',(#10213),#5899,.F.);
#95187=ADVANCED_FACE('',(#10214),#91279,.F.);
#95188=ADVANCED_FACE('',(#10215),#3186,.F.);
#95189=ADVANCED_FACE('',(#10216),#91280,.F.);
#95190=ADVANCED_FACE('',(#10217),#91281,.F.);
#95191=ADVANCED_FACE('',(#10218),#3187,.F.);
#95192=ADVANCED_FACE('',(#10219),#3188,.F.);
#95193=ADVANCED_FACE('',(#10220),#91282,.F.);
#95194=ADVANCED_FACE('',(#10221),#91283,.F.);
#95195=ADVANCED_FACE('',(#10222),#3189,.F.);
#95196=ADVANCED_FACE('',(#10223),#91284,.F.);
#95197=ADVANCED_FACE('',(#10224),#91285,.F.);
#95198=ADVANCED_FACE('',(#10225),#3190,.F.);
#95199=ADVANCED_FACE('',(#10226),#91286,.F.);
#95200=ADVANCED_FACE('',(#10227),#91287,.F.);
#95201=ADVANCED_FACE('',(#10228),#3191,.F.);
#95202=ADVANCED_FACE('',(#10229),#3192,.F.);
#95203=ADVANCED_FACE('',(#10230),#91288,.F.);
#95204=ADVANCED_FACE('',(#10231),#91289,.F.);
#95205=ADVANCED_FACE('',(#10232),#3193,.F.);
#95206=ADVANCED_FACE('',(#10233),#91290,.F.);
#95207=ADVANCED_FACE('',(#10234),#5900,.F.);
#95208=ADVANCED_FACE('',(#10235),#3194,.F.);
#95209=ADVANCED_FACE('',(#10236),#3195,.F.);
#95210=ADVANCED_FACE('',(#10237),#91291,.F.);
#95211=ADVANCED_FACE('',(#10238),#91292,.F.);
#95212=ADVANCED_FACE('',(#10239),#3196,.F.);
#95213=ADVANCED_FACE('',(#10240),#3197,.F.);
#95214=ADVANCED_FACE('',(#10241),#5901,.F.);
#95215=ADVANCED_FACE('',(#10242),#91293,.F.);
#95216=ADVANCED_FACE('',(#10243),#3198,.F.);
#95217=ADVANCED_FACE('',(#10244),#91294,.F.);
#95218=ADVANCED_FACE('',(#10245),#91295,.F.);
#95219=ADVANCED_FACE('',(#10246),#3199,.F.);
#95220=ADVANCED_FACE('',(#10247),#3200,.F.);
#95221=ADVANCED_FACE('',(#10248),#91296,.F.);
#95222=ADVANCED_FACE('',(#10249),#91297,.F.);
#95223=ADVANCED_FACE('',(#10250),#3201,.F.);
#95224=ADVANCED_FACE('',(#10251),#91298,.F.);
#95225=ADVANCED_FACE('',(#10252),#91299,.F.);
#95226=ADVANCED_FACE('',(#10253),#3202,.F.);
#95227=ADVANCED_FACE('',(#10254),#91300,.F.);
#95228=ADVANCED_FACE('',(#10255),#91301,.F.);
#95229=ADVANCED_FACE('',(#10256),#3203,.F.);
#95230=ADVANCED_FACE('',(#10257),#3204,.F.);
#95231=ADVANCED_FACE('',(#10258),#91302,.F.);
#95232=ADVANCED_FACE('',(#10259),#91303,.F.);
#95233=ADVANCED_FACE('',(#10260),#3205,.F.);
#95234=ADVANCED_FACE('',(#10261),#91304,.F.);
#95235=ADVANCED_FACE('',(#10262),#5902,.F.);
#95236=ADVANCED_FACE('',(#10263),#3206,.F.);
#95237=ADVANCED_FACE('',(#10264),#3207,.F.);
#95238=ADVANCED_FACE('',(#10265),#91305,.F.);
#95239=ADVANCED_FACE('',(#10266),#91306,.F.);
#95240=ADVANCED_FACE('',(#10267),#3208,.F.);
#95241=ADVANCED_FACE('',(#10268),#3209,.F.);
#95242=ADVANCED_FACE('',(#10269),#5903,.F.);
#95243=ADVANCED_FACE('',(#10270),#91307,.F.);
#95244=ADVANCED_FACE('',(#10271),#3210,.F.);
#95245=ADVANCED_FACE('',(#10272),#91308,.F.);
#95246=ADVANCED_FACE('',(#10273),#91309,.F.);
#95247=ADVANCED_FACE('',(#10274),#3211,.F.);
#95248=ADVANCED_FACE('',(#10275),#3212,.F.);
#95249=ADVANCED_FACE('',(#10276),#91310,.F.);
#95250=ADVANCED_FACE('',(#10277),#91311,.F.);
#95251=ADVANCED_FACE('',(#10278),#3213,.F.);
#95252=ADVANCED_FACE('',(#10279),#91312,.F.);
#95253=ADVANCED_FACE('',(#10280),#91313,.F.);
#95254=ADVANCED_FACE('',(#10281),#3214,.F.);
#95255=ADVANCED_FACE('',(#10282),#91314,.F.);
#95256=ADVANCED_FACE('',(#10283),#91315,.F.);
#95257=ADVANCED_FACE('',(#10284),#3215,.F.);
#95258=ADVANCED_FACE('',(#10285),#3216,.F.);
#95259=ADVANCED_FACE('',(#10286),#91316,.F.);
#95260=ADVANCED_FACE('',(#10287),#91317,.F.);
#95261=ADVANCED_FACE('',(#10288),#3217,.F.);
#95262=ADVANCED_FACE('',(#10289),#91318,.F.);
#95263=ADVANCED_FACE('',(#10290),#5904,.F.);
#95264=ADVANCED_FACE('',(#10291),#3218,.F.);
#95265=ADVANCED_FACE('',(#10292),#3219,.F.);
#95266=ADVANCED_FACE('',(#10293),#91319,.F.);
#95267=ADVANCED_FACE('',(#10294),#91320,.F.);
#95268=ADVANCED_FACE('',(#10295),#3220,.F.);
#95269=ADVANCED_FACE('',(#10296),#3221,.F.);
#95270=ADVANCED_FACE('',(#10297),#5905,.F.);
#95271=ADVANCED_FACE('',(#10298),#91321,.F.);
#95272=ADVANCED_FACE('',(#10299),#3222,.F.);
#95273=ADVANCED_FACE('',(#10300),#91322,.F.);
#95274=ADVANCED_FACE('',(#10301),#91323,.F.);
#95275=ADVANCED_FACE('',(#10302),#3223,.F.);
#95276=ADVANCED_FACE('',(#10303),#3224,.F.);
#95277=ADVANCED_FACE('',(#10304),#91324,.F.);
#95278=ADVANCED_FACE('',(#10305),#91325,.F.);
#95279=ADVANCED_FACE('',(#10306),#3225,.F.);
#95280=ADVANCED_FACE('',(#10307),#91326,.F.);
#95281=ADVANCED_FACE('',(#10308),#5906,.F.);
#95282=ADVANCED_FACE('',(#10309),#5907,.F.);
#95283=ADVANCED_FACE('',(#10310),#5908,.F.);
#95284=ADVANCED_FACE('',(#10311),#5909,.F.);
#95285=ADVANCED_FACE('',(#10312),#5910,.T.);
#95286=ADVANCED_FACE('',(#10313),#5911,.T.);
#95287=ADVANCED_FACE('',(#10314),#5912,.T.);
#95288=ADVANCED_FACE('',(#10315),#5913,.T.);
#95289=ADVANCED_FACE('',(#10316),#91327,.T.);
#95290=ADVANCED_FACE('',(#10317),#188,.T.);
#95291=ADVANCED_FACE('',(#10318),#189,.F.);
#95292=ADVANCED_FACE('',(#10319),#190,.T.);
#95293=ADVANCED_FACE('',(#10320),#191,.F.);
#95294=ADVANCED_FACE('',(#10321),#91328,.F.);
#95295=ADVANCED_FACE('',(#10322),#6865,.F.);
#95296=ADVANCED_FACE('',(#10323),#192,.F.);
#95297=ADVANCED_FACE('',(#10324),#6866,.F.);
#95298=ADVANCED_FACE('',(#10325),#193,.T.);
#95299=ADVANCED_FACE('',(#10326),#6867,.F.);
#95300=ADVANCED_FACE('',(#10327),#5914,.F.);
#95301=ADVANCED_FACE('',(#10328),#5915,.F.);
#95302=ADVANCED_FACE('',(#10329),#5916,.T.);
#95303=ADVANCED_FACE('',(#10330),#5917,.T.);
#95304=ADVANCED_FACE('',(#10331),#6868,.F.);
#95305=ADVANCED_FACE('',(#10332),#194,.F.);
#95306=ADVANCED_FACE('',(#10333),#6869,.F.);
#95307=ADVANCED_FACE('',(#10334),#195,.T.);
#95308=ADVANCED_FACE('',(#10335),#6870,.F.);
#95309=ADVANCED_FACE('',(#10336),#5918,.F.);
#95310=ADVANCED_FACE('',(#10337),#5919,.F.);
#95311=ADVANCED_FACE('',(#10338),#5920,.T.);
#95312=ADVANCED_FACE('',(#10339),#5921,.T.);
#95313=ADVANCED_FACE('',(#10340),#6871,.F.);
#95314=ADVANCED_FACE('',(#10341),#196,.F.);
#95315=ADVANCED_FACE('',(#10342),#6872,.F.);
#95316=ADVANCED_FACE('',(#10343),#197,.T.);
#95317=ADVANCED_FACE('',(#10344),#6873,.F.);
#95318=ADVANCED_FACE('',(#10345),#5922,.F.);
#95319=ADVANCED_FACE('',(#10346),#5923,.F.);
#95320=ADVANCED_FACE('',(#10347),#5924,.T.);
#95321=ADVANCED_FACE('',(#10348),#5925,.T.);
#95322=ADVANCED_FACE('',(#10349),#6874,.F.);
#95323=ADVANCED_FACE('',(#10350),#198,.F.);
#95324=ADVANCED_FACE('',(#10351),#6875,.F.);
#95325=ADVANCED_FACE('',(#10352),#199,.T.);
#95326=ADVANCED_FACE('',(#10353),#6876,.F.);
#95327=ADVANCED_FACE('',(#10354),#5926,.F.);
#95328=ADVANCED_FACE('',(#10355),#5927,.F.);
#95329=ADVANCED_FACE('',(#10356),#5928,.T.);
#95330=ADVANCED_FACE('',(#10357),#5929,.T.);
#95331=ADVANCED_FACE('',(#10358),#6877,.F.);
#95332=ADVANCED_FACE('',(#10359),#200,.F.);
#95333=ADVANCED_FACE('',(#10360),#6878,.F.);
#95334=ADVANCED_FACE('',(#10361),#201,.T.);
#95335=ADVANCED_FACE('',(#10362),#6879,.F.);
#95336=ADVANCED_FACE('',(#10363),#5930,.F.);
#95337=ADVANCED_FACE('',(#10364),#5931,.F.);
#95338=ADVANCED_FACE('',(#10365),#5932,.T.);
#95339=ADVANCED_FACE('',(#10366),#5933,.T.);
#95340=ADVANCED_FACE('',(#10367),#6880,.F.);
#95341=ADVANCED_FACE('',(#10368),#202,.F.);
#95342=ADVANCED_FACE('',(#10369),#6881,.F.);
#95343=ADVANCED_FACE('',(#10370),#203,.T.);
#95344=ADVANCED_FACE('',(#10371),#6882,.F.);
#95345=ADVANCED_FACE('',(#10372),#5934,.F.);
#95346=ADVANCED_FACE('',(#10373),#5935,.F.);
#95347=ADVANCED_FACE('',(#10374),#5936,.T.);
#95348=ADVANCED_FACE('',(#10375),#5937,.T.);
#95349=ADVANCED_FACE('',(#10376),#6883,.F.);
#95350=ADVANCED_FACE('',(#10377),#204,.F.);
#95351=ADVANCED_FACE('',(#10378),#6884,.F.);
#95352=ADVANCED_FACE('',(#10379),#205,.T.);
#95353=ADVANCED_FACE('',(#10380),#6885,.F.);
#95354=ADVANCED_FACE('',(#10381),#5938,.F.);
#95355=ADVANCED_FACE('',(#10382),#5939,.F.);
#95356=ADVANCED_FACE('',(#10383),#5940,.T.);
#95357=ADVANCED_FACE('',(#10384),#5941,.T.);
#95358=ADVANCED_FACE('',(#10385),#6886,.F.);
#95359=ADVANCED_FACE('',(#10386),#206,.F.);
#95360=ADVANCED_FACE('',(#10387),#6887,.F.);
#95361=ADVANCED_FACE('',(#10388),#207,.T.);
#95362=ADVANCED_FACE('',(#10389),#6888,.F.);
#95363=ADVANCED_FACE('',(#10390),#5942,.F.);
#95364=ADVANCED_FACE('',(#10391),#5943,.F.);
#95365=ADVANCED_FACE('',(#10392),#5944,.T.);
#95366=ADVANCED_FACE('',(#10393),#5945,.T.);
#95367=ADVANCED_FACE('',(#10394),#6889,.F.);
#95368=ADVANCED_FACE('',(#10395),#208,.F.);
#95369=ADVANCED_FACE('',(#10396),#6890,.F.);
#95370=ADVANCED_FACE('',(#10397),#209,.T.);
#95371=ADVANCED_FACE('',(#10398),#6891,.F.);
#95372=ADVANCED_FACE('',(#10399),#5946,.F.);
#95373=ADVANCED_FACE('',(#10400),#5947,.F.);
#95374=ADVANCED_FACE('',(#10401),#5948,.T.);
#95375=ADVANCED_FACE('',(#10402),#5949,.T.);
#95376=ADVANCED_FACE('',(#10403),#6892,.F.);
#95377=ADVANCED_FACE('',(#10404),#210,.F.);
#95378=ADVANCED_FACE('',(#10405),#6893,.F.);
#95379=ADVANCED_FACE('',(#10406),#211,.T.);
#95380=ADVANCED_FACE('',(#10407),#6894,.F.);
#95381=ADVANCED_FACE('',(#10408),#5950,.F.);
#95382=ADVANCED_FACE('',(#10409),#5951,.F.);
#95383=ADVANCED_FACE('',(#10410),#5952,.T.);
#95384=ADVANCED_FACE('',(#10411),#5953,.T.);
#95385=ADVANCED_FACE('',(#10412),#6895,.F.);
#95386=ADVANCED_FACE('',(#10413),#212,.F.);
#95387=ADVANCED_FACE('',(#10414),#6896,.F.);
#95388=ADVANCED_FACE('',(#10415),#213,.T.);
#95389=ADVANCED_FACE('',(#10416),#6897,.F.);
#95390=ADVANCED_FACE('',(#10417),#5954,.F.);
#95391=ADVANCED_FACE('',(#10418),#5955,.F.);
#95392=ADVANCED_FACE('',(#10419),#5956,.T.);
#95393=ADVANCED_FACE('',(#10420),#5957,.T.);
#95394=ADVANCED_FACE('',(#10421),#6898,.F.);
#95395=ADVANCED_FACE('',(#10422),#214,.F.);
#95396=ADVANCED_FACE('',(#10423),#6899,.F.);
#95397=ADVANCED_FACE('',(#10424),#215,.T.);
#95398=ADVANCED_FACE('',(#10425),#6900,.F.);
#95399=ADVANCED_FACE('',(#10426),#5958,.F.);
#95400=ADVANCED_FACE('',(#10427),#5959,.F.);
#95401=ADVANCED_FACE('',(#10428),#5960,.T.);
#95402=ADVANCED_FACE('',(#10429),#5961,.T.);
#95403=ADVANCED_FACE('',(#10430),#6901,.F.);
#95404=ADVANCED_FACE('',(#10431),#216,.F.);
#95405=ADVANCED_FACE('',(#10432),#6902,.F.);
#95406=ADVANCED_FACE('',(#10433),#217,.T.);
#95407=ADVANCED_FACE('',(#10434),#6903,.F.);
#95408=ADVANCED_FACE('',(#10435),#5962,.F.);
#95409=ADVANCED_FACE('',(#10436),#5963,.F.);
#95410=ADVANCED_FACE('',(#10437),#5964,.T.);
#95411=ADVANCED_FACE('',(#10438),#5965,.T.);
#95412=ADVANCED_FACE('',(#10439),#6904,.F.);
#95413=ADVANCED_FACE('',(#10440),#218,.F.);
#95414=ADVANCED_FACE('',(#10441),#6905,.F.);
#95415=ADVANCED_FACE('',(#10442),#219,.T.);
#95416=ADVANCED_FACE('',(#10443),#6906,.F.);
#95417=ADVANCED_FACE('',(#10444),#5966,.F.);
#95418=ADVANCED_FACE('',(#10445),#5967,.F.);
#95419=ADVANCED_FACE('',(#10446),#5968,.T.);
#95420=ADVANCED_FACE('',(#10447),#5969,.T.);
#95421=ADVANCED_FACE('',(#10448),#6907,.F.);
#95422=ADVANCED_FACE('',(#10449),#220,.F.);
#95423=ADVANCED_FACE('',(#10450),#6908,.F.);
#95424=ADVANCED_FACE('',(#10451),#221,.T.);
#95425=ADVANCED_FACE('',(#10452),#6909,.F.);
#95426=ADVANCED_FACE('',(#10453),#5970,.F.);
#95427=ADVANCED_FACE('',(#10454),#5971,.F.);
#95428=ADVANCED_FACE('',(#10455),#5972,.T.);
#95429=ADVANCED_FACE('',(#10456),#5973,.T.);
#95430=ADVANCED_FACE('',(#10457),#6910,.F.);
#95431=ADVANCED_FACE('',(#10458),#222,.F.);
#95432=ADVANCED_FACE('',(#10459),#6911,.F.);
#95433=ADVANCED_FACE('',(#10460),#223,.T.);
#95434=ADVANCED_FACE('',(#10461),#6912,.F.);
#95435=ADVANCED_FACE('',(#10462),#5974,.F.);
#95436=ADVANCED_FACE('',(#10463),#5975,.F.);
#95437=ADVANCED_FACE('',(#10464),#5976,.T.);
#95438=ADVANCED_FACE('',(#10465),#5977,.T.);
#95439=ADVANCED_FACE('',(#10466),#6913,.F.);
#95440=ADVANCED_FACE('',(#10467),#224,.F.);
#95441=ADVANCED_FACE('',(#10468),#6914,.F.);
#95442=ADVANCED_FACE('',(#10469),#225,.T.);
#95443=ADVANCED_FACE('',(#10470),#6915,.F.);
#95444=ADVANCED_FACE('',(#10471),#5978,.F.);
#95445=ADVANCED_FACE('',(#10472),#5979,.F.);
#95446=ADVANCED_FACE('',(#10473),#5980,.T.);
#95447=ADVANCED_FACE('',(#10474),#5981,.T.);
#95448=ADVANCED_FACE('',(#10475),#6916,.F.);
#95449=ADVANCED_FACE('',(#10476),#226,.F.);
#95450=ADVANCED_FACE('',(#10477),#6917,.F.);
#95451=ADVANCED_FACE('',(#10478),#227,.T.);
#95452=ADVANCED_FACE('',(#10479),#6918,.F.);
#95453=ADVANCED_FACE('',(#10480),#5982,.F.);
#95454=ADVANCED_FACE('',(#10481),#5983,.F.);
#95455=ADVANCED_FACE('',(#10482),#5984,.T.);
#95456=ADVANCED_FACE('',(#10483),#5985,.T.);
#95457=ADVANCED_FACE('',(#10484),#6919,.F.);
#95458=ADVANCED_FACE('',(#10485),#228,.F.);
#95459=ADVANCED_FACE('',(#10486),#6920,.F.);
#95460=ADVANCED_FACE('',(#10487),#229,.T.);
#95461=ADVANCED_FACE('',(#10488),#6921,.F.);
#95462=ADVANCED_FACE('',(#10489),#5986,.F.);
#95463=ADVANCED_FACE('',(#10490),#5987,.F.);
#95464=ADVANCED_FACE('',(#10491),#5988,.T.);
#95465=ADVANCED_FACE('',(#10492),#5989,.T.);
#95466=ADVANCED_FACE('',(#10493),#6922,.F.);
#95467=ADVANCED_FACE('',(#10494),#230,.F.);
#95468=ADVANCED_FACE('',(#10495),#6923,.F.);
#95469=ADVANCED_FACE('',(#10496),#231,.T.);
#95470=ADVANCED_FACE('',(#10497),#6924,.F.);
#95471=ADVANCED_FACE('',(#10498),#5990,.F.);
#95472=ADVANCED_FACE('',(#10499),#5991,.F.);
#95473=ADVANCED_FACE('',(#10500),#5992,.T.);
#95474=ADVANCED_FACE('',(#10501),#5993,.T.);
#95475=ADVANCED_FACE('',(#10502),#6925,.F.);
#95476=ADVANCED_FACE('',(#10503),#232,.F.);
#95477=ADVANCED_FACE('',(#10504),#6926,.F.);
#95478=ADVANCED_FACE('',(#10505),#233,.T.);
#95479=ADVANCED_FACE('',(#10506),#6927,.F.);
#95480=ADVANCED_FACE('',(#10507),#5994,.F.);
#95481=ADVANCED_FACE('',(#10508),#5995,.F.);
#95482=ADVANCED_FACE('',(#10509),#5996,.T.);
#95483=ADVANCED_FACE('',(#10510),#5997,.T.);
#95484=ADVANCED_FACE('',(#10511),#6928,.F.);
#95485=ADVANCED_FACE('',(#10512),#234,.F.);
#95486=ADVANCED_FACE('',(#10513),#6929,.F.);
#95487=ADVANCED_FACE('',(#10514),#235,.T.);
#95488=ADVANCED_FACE('',(#10515),#6930,.F.);
#95489=ADVANCED_FACE('',(#10516),#5998,.F.);
#95490=ADVANCED_FACE('',(#10517),#5999,.F.);
#95491=ADVANCED_FACE('',(#10518),#6000,.T.);
#95492=ADVANCED_FACE('',(#10519),#6001,.T.);
#95493=ADVANCED_FACE('',(#10520),#6931,.F.);
#95494=ADVANCED_FACE('',(#10521),#236,.F.);
#95495=ADVANCED_FACE('',(#10522),#6932,.F.);
#95496=ADVANCED_FACE('',(#10523),#237,.T.);
#95497=ADVANCED_FACE('',(#10524),#6933,.F.);
#95498=ADVANCED_FACE('',(#10525),#6002,.F.);
#95499=ADVANCED_FACE('',(#10526),#6003,.F.);
#95500=ADVANCED_FACE('',(#10527),#6004,.T.);
#95501=ADVANCED_FACE('',(#10528),#6005,.T.);
#95502=ADVANCED_FACE('',(#10529),#6934,.F.);
#95503=ADVANCED_FACE('',(#10530),#238,.F.);
#95504=ADVANCED_FACE('',(#10531),#6935,.F.);
#95505=ADVANCED_FACE('',(#10532),#239,.T.);
#95506=ADVANCED_FACE('',(#10533),#6936,.F.);
#95507=ADVANCED_FACE('',(#10534),#6006,.F.);
#95508=ADVANCED_FACE('',(#10535),#6007,.F.);
#95509=ADVANCED_FACE('',(#10536),#6008,.T.);
#95510=ADVANCED_FACE('',(#10537),#6009,.T.);
#95511=ADVANCED_FACE('',(#10538),#6937,.F.);
#95512=ADVANCED_FACE('',(#10539),#240,.F.);
#95513=ADVANCED_FACE('',(#10540),#6938,.F.);
#95514=ADVANCED_FACE('',(#10541),#241,.T.);
#95515=ADVANCED_FACE('',(#10542),#6939,.F.);
#95516=ADVANCED_FACE('',(#10543),#6010,.F.);
#95517=ADVANCED_FACE('',(#10544),#6011,.F.);
#95518=ADVANCED_FACE('',(#10545),#6012,.T.);
#95519=ADVANCED_FACE('',(#10546),#6013,.T.);
#95520=ADVANCED_FACE('',(#10547),#6940,.F.);
#95521=ADVANCED_FACE('',(#10548),#242,.F.);
#95522=ADVANCED_FACE('',(#10549),#6941,.F.);
#95523=ADVANCED_FACE('',(#10550),#243,.T.);
#95524=ADVANCED_FACE('',(#10551),#6942,.F.);
#95525=ADVANCED_FACE('',(#10552),#6014,.F.);
#95526=ADVANCED_FACE('',(#10553),#6015,.F.);
#95527=ADVANCED_FACE('',(#10554),#6016,.T.);
#95528=ADVANCED_FACE('',(#10555),#6017,.T.);
#95529=ADVANCED_FACE('',(#10556),#6943,.F.);
#95530=ADVANCED_FACE('',(#10557),#244,.F.);
#95531=ADVANCED_FACE('',(#10558),#6944,.F.);
#95532=ADVANCED_FACE('',(#10559),#245,.T.);
#95533=ADVANCED_FACE('',(#10560),#6945,.F.);
#95534=ADVANCED_FACE('',(#10561),#6018,.F.);
#95535=ADVANCED_FACE('',(#10562),#6019,.F.);
#95536=ADVANCED_FACE('',(#10563),#6020,.T.);
#95537=ADVANCED_FACE('',(#10564),#6021,.T.);
#95538=ADVANCED_FACE('',(#10565),#6946,.F.);
#95539=ADVANCED_FACE('',(#10566),#246,.F.);
#95540=ADVANCED_FACE('',(#10567),#6947,.F.);
#95541=ADVANCED_FACE('',(#10568),#247,.T.);
#95542=ADVANCED_FACE('',(#10569),#6948,.F.);
#95543=ADVANCED_FACE('',(#10570),#6022,.F.);
#95544=ADVANCED_FACE('',(#10571),#6023,.F.);
#95545=ADVANCED_FACE('',(#10572),#6024,.T.);
#95546=ADVANCED_FACE('',(#10573),#6025,.T.);
#95547=ADVANCED_FACE('',(#10574),#6949,.F.);
#95548=ADVANCED_FACE('',(#10575),#248,.F.);
#95549=ADVANCED_FACE('',(#10576),#6950,.F.);
#95550=ADVANCED_FACE('',(#10577),#249,.T.);
#95551=ADVANCED_FACE('',(#10578),#6951,.F.);
#95552=ADVANCED_FACE('',(#10579),#6026,.F.);
#95553=ADVANCED_FACE('',(#10580),#6027,.F.);
#95554=ADVANCED_FACE('',(#10581),#6028,.T.);
#95555=ADVANCED_FACE('',(#10582),#6029,.T.);
#95556=ADVANCED_FACE('',(#10583),#6952,.F.);
#95557=ADVANCED_FACE('',(#10584),#250,.F.);
#95558=ADVANCED_FACE('',(#10585),#6953,.F.);
#95559=ADVANCED_FACE('',(#10586),#251,.T.);
#95560=ADVANCED_FACE('',(#10587),#6954,.F.);
#95561=ADVANCED_FACE('',(#10588),#6030,.F.);
#95562=ADVANCED_FACE('',(#10589),#6031,.F.);
#95563=ADVANCED_FACE('',(#10590),#6032,.T.);
#95564=ADVANCED_FACE('',(#10591),#6033,.T.);
#95565=ADVANCED_FACE('',(#10592),#6955,.F.);
#95566=ADVANCED_FACE('',(#10593),#252,.F.);
#95567=ADVANCED_FACE('',(#10594),#6956,.F.);
#95568=ADVANCED_FACE('',(#10595),#253,.T.);
#95569=ADVANCED_FACE('',(#10596),#6957,.F.);
#95570=ADVANCED_FACE('',(#10597),#6034,.F.);
#95571=ADVANCED_FACE('',(#10598),#6035,.F.);
#95572=ADVANCED_FACE('',(#10599),#6036,.T.);
#95573=ADVANCED_FACE('',(#10600),#6037,.T.);
#95574=ADVANCED_FACE('',(#10601),#6958,.F.);
#95575=ADVANCED_FACE('',(#10602),#254,.F.);
#95576=ADVANCED_FACE('',(#10603),#6959,.F.);
#95577=ADVANCED_FACE('',(#10604),#255,.T.);
#95578=ADVANCED_FACE('',(#10605),#6960,.F.);
#95579=ADVANCED_FACE('',(#10606),#6038,.F.);
#95580=ADVANCED_FACE('',(#10607),#6039,.F.);
#95581=ADVANCED_FACE('',(#10608),#6040,.T.);
#95582=ADVANCED_FACE('',(#10609),#6041,.T.);
#95583=ADVANCED_FACE('',(#10610),#6961,.F.);
#95584=ADVANCED_FACE('',(#10611),#256,.F.);
#95585=ADVANCED_FACE('',(#10612),#6962,.F.);
#95586=ADVANCED_FACE('',(#10613),#257,.T.);
#95587=ADVANCED_FACE('',(#10614),#6963,.F.);
#95588=ADVANCED_FACE('',(#10615),#6042,.F.);
#95589=ADVANCED_FACE('',(#10616),#6043,.F.);
#95590=ADVANCED_FACE('',(#10617),#6044,.T.);
#95591=ADVANCED_FACE('',(#10618),#6045,.T.);
#95592=ADVANCED_FACE('',(#10619),#6964,.F.);
#95593=ADVANCED_FACE('',(#10620),#258,.F.);
#95594=ADVANCED_FACE('',(#10621),#6965,.F.);
#95595=ADVANCED_FACE('',(#10622),#259,.T.);
#95596=ADVANCED_FACE('',(#10623),#6966,.F.);
#95597=ADVANCED_FACE('',(#10624),#6046,.F.);
#95598=ADVANCED_FACE('',(#10625),#6047,.F.);
#95599=ADVANCED_FACE('',(#10626),#6048,.T.);
#95600=ADVANCED_FACE('',(#10627),#6049,.T.);
#95601=ADVANCED_FACE('',(#10628),#6967,.F.);
#95602=ADVANCED_FACE('',(#10629),#260,.F.);
#95603=ADVANCED_FACE('',(#10630),#6968,.F.);
#95604=ADVANCED_FACE('',(#10631),#261,.T.);
#95605=ADVANCED_FACE('',(#10632),#6969,.F.);
#95606=ADVANCED_FACE('',(#10633),#6050,.F.);
#95607=ADVANCED_FACE('',(#10634),#6051,.F.);
#95608=ADVANCED_FACE('',(#10635),#6052,.T.);
#95609=ADVANCED_FACE('',(#10636),#6053,.T.);
#95610=ADVANCED_FACE('',(#10637),#6970,.F.);
#95611=ADVANCED_FACE('',(#10638),#262,.F.);
#95612=ADVANCED_FACE('',(#10639),#6971,.F.);
#95613=ADVANCED_FACE('',(#10640),#263,.T.);
#95614=ADVANCED_FACE('',(#10641),#6972,.F.);
#95615=ADVANCED_FACE('',(#10642),#6054,.F.);
#95616=ADVANCED_FACE('',(#10643),#6055,.F.);
#95617=ADVANCED_FACE('',(#10644),#6056,.T.);
#95618=ADVANCED_FACE('',(#10645),#6057,.T.);
#95619=ADVANCED_FACE('',(#10646),#6973,.F.);
#95620=ADVANCED_FACE('',(#10647),#264,.F.);
#95621=ADVANCED_FACE('',(#10648),#6974,.F.);
#95622=ADVANCED_FACE('',(#10649),#265,.T.);
#95623=ADVANCED_FACE('',(#10650),#6975,.F.);
#95624=ADVANCED_FACE('',(#10651),#6058,.F.);
#95625=ADVANCED_FACE('',(#10652),#6059,.F.);
#95626=ADVANCED_FACE('',(#10653),#6060,.T.);
#95627=ADVANCED_FACE('',(#10654),#6061,.T.);
#95628=ADVANCED_FACE('',(#10655),#6976,.F.);
#95629=ADVANCED_FACE('',(#10656),#266,.F.);
#95630=ADVANCED_FACE('',(#10657),#6977,.F.);
#95631=ADVANCED_FACE('',(#10658),#267,.T.);
#95632=ADVANCED_FACE('',(#10659),#6978,.F.);
#95633=ADVANCED_FACE('',(#10660),#6062,.F.);
#95634=ADVANCED_FACE('',(#10661),#6063,.F.);
#95635=ADVANCED_FACE('',(#10662),#6064,.T.);
#95636=ADVANCED_FACE('',(#10663),#6065,.T.);
#95637=ADVANCED_FACE('',(#10664),#6979,.F.);
#95638=ADVANCED_FACE('',(#10665),#268,.F.);
#95639=ADVANCED_FACE('',(#10666),#6980,.F.);
#95640=ADVANCED_FACE('',(#10667),#269,.T.);
#95641=ADVANCED_FACE('',(#10668),#6981,.F.);
#95642=ADVANCED_FACE('',(#10669),#6066,.F.);
#95643=ADVANCED_FACE('',(#10670),#6067,.F.);
#95644=ADVANCED_FACE('',(#10671),#6068,.T.);
#95645=ADVANCED_FACE('',(#10672),#6069,.T.);
#95646=ADVANCED_FACE('',(#10673),#6982,.F.);
#95647=ADVANCED_FACE('',(#10674),#270,.F.);
#95648=ADVANCED_FACE('',(#10675),#6983,.F.);
#95649=ADVANCED_FACE('',(#10676),#271,.T.);
#95650=ADVANCED_FACE('',(#10677),#6984,.F.);
#95651=ADVANCED_FACE('',(#10678),#6070,.F.);
#95652=ADVANCED_FACE('',(#10679),#6071,.F.);
#95653=ADVANCED_FACE('',(#10680),#6072,.T.);
#95654=ADVANCED_FACE('',(#10681),#6073,.T.);
#95655=ADVANCED_FACE('',(#10682),#6985,.F.);
#95656=ADVANCED_FACE('',(#10683),#272,.F.);
#95657=ADVANCED_FACE('',(#10684),#6986,.F.);
#95658=ADVANCED_FACE('',(#10685),#273,.T.);
#95659=ADVANCED_FACE('',(#10686),#6987,.F.);
#95660=ADVANCED_FACE('',(#10687),#6074,.F.);
#95661=ADVANCED_FACE('',(#10688),#6075,.F.);
#95662=ADVANCED_FACE('',(#10689),#6076,.T.);
#95663=ADVANCED_FACE('',(#10690),#6077,.T.);
#95664=ADVANCED_FACE('',(#10691),#6988,.F.);
#95665=ADVANCED_FACE('',(#10692),#274,.F.);
#95666=ADVANCED_FACE('',(#10693),#6989,.F.);
#95667=ADVANCED_FACE('',(#10694),#275,.T.);
#95668=ADVANCED_FACE('',(#10695),#6990,.F.);
#95669=ADVANCED_FACE('',(#10696),#6078,.F.);
#95670=ADVANCED_FACE('',(#10697),#6079,.F.);
#95671=ADVANCED_FACE('',(#10698),#6080,.T.);
#95672=ADVANCED_FACE('',(#10699),#6081,.T.);
#95673=ADVANCED_FACE('',(#10700),#6991,.F.);
#95674=ADVANCED_FACE('',(#10701),#276,.F.);
#95675=ADVANCED_FACE('',(#10702),#6992,.F.);
#95676=ADVANCED_FACE('',(#10703),#277,.T.);
#95677=ADVANCED_FACE('',(#10704),#6993,.F.);
#95678=ADVANCED_FACE('',(#10705),#6082,.F.);
#95679=ADVANCED_FACE('',(#10706),#6083,.F.);
#95680=ADVANCED_FACE('',(#10707),#6084,.T.);
#95681=ADVANCED_FACE('',(#10708),#6085,.T.);
#95682=ADVANCED_FACE('',(#10709),#6994,.F.);
#95683=ADVANCED_FACE('',(#10710),#278,.F.);
#95684=ADVANCED_FACE('',(#10711),#6995,.F.);
#95685=ADVANCED_FACE('',(#10712),#279,.T.);
#95686=ADVANCED_FACE('',(#10713),#6996,.F.);
#95687=ADVANCED_FACE('',(#10714),#6086,.F.);
#95688=ADVANCED_FACE('',(#10715),#6087,.F.);
#95689=ADVANCED_FACE('',(#10716),#6088,.T.);
#95690=ADVANCED_FACE('',(#10717),#6089,.T.);
#95691=ADVANCED_FACE('',(#10718),#6997,.F.);
#95692=ADVANCED_FACE('',(#10719),#280,.F.);
#95693=ADVANCED_FACE('',(#10720),#6998,.F.);
#95694=ADVANCED_FACE('',(#10721),#281,.T.);
#95695=ADVANCED_FACE('',(#10722),#6999,.F.);
#95696=ADVANCED_FACE('',(#10723),#6090,.F.);
#95697=ADVANCED_FACE('',(#10724),#6091,.F.);
#95698=ADVANCED_FACE('',(#10725),#6092,.T.);
#95699=ADVANCED_FACE('',(#10726),#6093,.T.);
#95700=ADVANCED_FACE('',(#10727),#7000,.F.);
#95701=ADVANCED_FACE('',(#10728),#282,.F.);
#95702=ADVANCED_FACE('',(#10729),#7001,.F.);
#95703=ADVANCED_FACE('',(#10730),#283,.T.);
#95704=ADVANCED_FACE('',(#10731),#7002,.F.);
#95705=ADVANCED_FACE('',(#10732),#6094,.F.);
#95706=ADVANCED_FACE('',(#10733),#6095,.F.);
#95707=ADVANCED_FACE('',(#10734),#6096,.T.);
#95708=ADVANCED_FACE('',(#10735),#6097,.T.);
#95709=ADVANCED_FACE('',(#10736),#7003,.F.);
#95710=ADVANCED_FACE('',(#10737),#284,.F.);
#95711=ADVANCED_FACE('',(#10738),#7004,.F.);
#95712=ADVANCED_FACE('',(#10739),#285,.T.);
#95713=ADVANCED_FACE('',(#10740),#7005,.F.);
#95714=ADVANCED_FACE('',(#10741),#6098,.F.);
#95715=ADVANCED_FACE('',(#10742),#6099,.F.);
#95716=ADVANCED_FACE('',(#10743),#6100,.T.);
#95717=ADVANCED_FACE('',(#10744),#6101,.T.);
#95718=ADVANCED_FACE('',(#10745),#7006,.F.);
#95719=ADVANCED_FACE('',(#10746),#286,.F.);
#95720=ADVANCED_FACE('',(#10747),#7007,.F.);
#95721=ADVANCED_FACE('',(#10748),#287,.T.);
#95722=ADVANCED_FACE('',(#10749),#7008,.F.);
#95723=ADVANCED_FACE('',(#10750),#6102,.F.);
#95724=ADVANCED_FACE('',(#10751),#6103,.F.);
#95725=ADVANCED_FACE('',(#10752),#6104,.T.);
#95726=ADVANCED_FACE('',(#10753),#6105,.T.);
#95727=ADVANCED_FACE('',(#10754),#7009,.F.);
#95728=ADVANCED_FACE('',(#10755),#288,.F.);
#95729=ADVANCED_FACE('',(#10756),#7010,.F.);
#95730=ADVANCED_FACE('',(#10757),#289,.T.);
#95731=ADVANCED_FACE('',(#10758),#7011,.F.);
#95732=ADVANCED_FACE('',(#10759),#6106,.F.);
#95733=ADVANCED_FACE('',(#10760),#6107,.F.);
#95734=ADVANCED_FACE('',(#10761),#6108,.T.);
#95735=ADVANCED_FACE('',(#10762),#6109,.T.);
#95736=ADVANCED_FACE('',(#10763),#7012,.F.);
#95737=ADVANCED_FACE('',(#10764),#290,.F.);
#95738=ADVANCED_FACE('',(#10765),#7013,.F.);
#95739=ADVANCED_FACE('',(#10766),#291,.T.);
#95740=ADVANCED_FACE('',(#10767),#7014,.F.);
#95741=ADVANCED_FACE('',(#10768),#6110,.F.);
#95742=ADVANCED_FACE('',(#10769),#6111,.F.);
#95743=ADVANCED_FACE('',(#10770),#6112,.T.);
#95744=ADVANCED_FACE('',(#10771),#6113,.T.);
#95745=ADVANCED_FACE('',(#10772),#7015,.F.);
#95746=ADVANCED_FACE('',(#10773),#292,.F.);
#95747=ADVANCED_FACE('',(#10774),#7016,.F.);
#95748=ADVANCED_FACE('',(#10775),#293,.T.);
#95749=ADVANCED_FACE('',(#10776),#7017,.F.);
#95750=ADVANCED_FACE('',(#10777),#6114,.F.);
#95751=ADVANCED_FACE('',(#10778),#6115,.F.);
#95752=ADVANCED_FACE('',(#10779),#6116,.T.);
#95753=ADVANCED_FACE('',(#10780),#6117,.T.);
#95754=ADVANCED_FACE('',(#10781),#7018,.F.);
#95755=ADVANCED_FACE('',(#10782),#294,.F.);
#95756=ADVANCED_FACE('',(#10783),#7019,.F.);
#95757=ADVANCED_FACE('',(#10784),#295,.T.);
#95758=ADVANCED_FACE('',(#10785),#7020,.F.);
#95759=ADVANCED_FACE('',(#10786),#6118,.F.);
#95760=ADVANCED_FACE('',(#10787),#6119,.F.);
#95761=ADVANCED_FACE('',(#10788),#6120,.T.);
#95762=ADVANCED_FACE('',(#10789),#6121,.T.);
#95763=ADVANCED_FACE('',(#10790),#7021,.F.);
#95764=ADVANCED_FACE('',(#10791),#296,.F.);
#95765=ADVANCED_FACE('',(#10792),#7022,.F.);
#95766=ADVANCED_FACE('',(#10793),#297,.T.);
#95767=ADVANCED_FACE('',(#10794),#7023,.F.);
#95768=ADVANCED_FACE('',(#10795),#6122,.F.);
#95769=ADVANCED_FACE('',(#10796),#6123,.F.);
#95770=ADVANCED_FACE('',(#10797),#6124,.T.);
#95771=ADVANCED_FACE('',(#10798),#6125,.T.);
#95772=ADVANCED_FACE('',(#10799),#7024,.F.);
#95773=ADVANCED_FACE('',(#10800),#298,.F.);
#95774=ADVANCED_FACE('',(#10801),#7025,.F.);
#95775=ADVANCED_FACE('',(#10802),#299,.T.);
#95776=ADVANCED_FACE('',(#10803),#7026,.F.);
#95777=ADVANCED_FACE('',(#10804),#6126,.F.);
#95778=ADVANCED_FACE('',(#10805),#6127,.F.);
#95779=ADVANCED_FACE('',(#10806),#6128,.T.);
#95780=ADVANCED_FACE('',(#10807),#6129,.T.);
#95781=ADVANCED_FACE('',(#10808),#7027,.F.);
#95782=ADVANCED_FACE('',(#10809),#300,.F.);
#95783=ADVANCED_FACE('',(#10810),#7028,.F.);
#95784=ADVANCED_FACE('',(#10811),#301,.T.);
#95785=ADVANCED_FACE('',(#10812),#7029,.F.);
#95786=ADVANCED_FACE('',(#10813),#6130,.F.);
#95787=ADVANCED_FACE('',(#10814),#6131,.F.);
#95788=ADVANCED_FACE('',(#10815),#6132,.T.);
#95789=ADVANCED_FACE('',(#10816),#6133,.T.);
#95790=ADVANCED_FACE('',(#10817),#7030,.F.);
#95791=ADVANCED_FACE('',(#10818),#302,.F.);
#95792=ADVANCED_FACE('',(#10819),#7031,.F.);
#95793=ADVANCED_FACE('',(#10820),#303,.T.);
#95794=ADVANCED_FACE('',(#10821),#7032,.F.);
#95795=ADVANCED_FACE('',(#10822),#6134,.F.);
#95796=ADVANCED_FACE('',(#10823),#6135,.F.);
#95797=ADVANCED_FACE('',(#10824),#6136,.T.);
#95798=ADVANCED_FACE('',(#10825),#6137,.T.);
#95799=ADVANCED_FACE('',(#10826),#7033,.F.);
#95800=ADVANCED_FACE('',(#10827),#304,.F.);
#95801=ADVANCED_FACE('',(#10828),#7034,.F.);
#95802=ADVANCED_FACE('',(#10829),#305,.T.);
#95803=ADVANCED_FACE('',(#10830),#7035,.F.);
#95804=ADVANCED_FACE('',(#10831),#6138,.F.);
#95805=ADVANCED_FACE('',(#10832),#6139,.F.);
#95806=ADVANCED_FACE('',(#10833),#6140,.T.);
#95807=ADVANCED_FACE('',(#10834),#6141,.T.);
#95808=ADVANCED_FACE('',(#10835),#7036,.F.);
#95809=ADVANCED_FACE('',(#10836),#306,.F.);
#95810=ADVANCED_FACE('',(#10837),#7037,.F.);
#95811=ADVANCED_FACE('',(#10838),#307,.T.);
#95812=ADVANCED_FACE('',(#10839),#7038,.F.);
#95813=ADVANCED_FACE('',(#10840),#6142,.F.);
#95814=ADVANCED_FACE('',(#10841),#6143,.F.);
#95815=ADVANCED_FACE('',(#10842),#6144,.T.);
#95816=ADVANCED_FACE('',(#10843),#6145,.T.);
#95817=ADVANCED_FACE('',(#10844),#7039,.F.);
#95818=ADVANCED_FACE('',(#10845),#308,.F.);
#95819=ADVANCED_FACE('',(#10846),#7040,.F.);
#95820=ADVANCED_FACE('',(#10847),#309,.T.);
#95821=ADVANCED_FACE('',(#10848),#7041,.F.);
#95822=ADVANCED_FACE('',(#10849),#6146,.F.);
#95823=ADVANCED_FACE('',(#10850),#6147,.F.);
#95824=ADVANCED_FACE('',(#10851),#6148,.T.);
#95825=ADVANCED_FACE('',(#10852),#6149,.T.);
#95826=ADVANCED_FACE('',(#10853,#6369),#7042,.F.);
#95827=ADVANCED_FACE('',(#10854),#7043,.F.);
#95828=ADVANCED_FACE('',(#10855),#310,.F.);
#95829=ADVANCED_FACE('',(#10856),#7044,.F.);
#95830=ADVANCED_FACE('',(#10857),#311,.T.);
#95831=ADVANCED_FACE('',(#10858),#7045,.F.);
#95832=ADVANCED_FACE('',(#10859,#6370),#7046,.F.);
#95833=ADVANCED_FACE('',(#10860,#6371),#7047,.F.);
#95834=ADVANCED_FACE('',(#10861),#6150,.F.);
#95835=ADVANCED_FACE('',(#10862),#6151,.F.);
#95836=ADVANCED_FACE('',(#10863),#6152,.T.);
#95837=ADVANCED_FACE('',(#10864),#6153,.T.);
#95838=ADVANCED_FACE('',(#10865),#7048,.F.);
#95839=ADVANCED_FACE('',(#10866),#7049,.T.);
#95840=ADVANCED_FACE('',(#10867),#7050,.F.);
#95841=ADVANCED_FACE('',(#10868),#91329,.T.);
#95842=ADVANCED_FACE('',(#10869),#91330,.T.);
#95843=ADVANCED_FACE('',(#10870),#91331,.F.);
#95844=ADVANCED_FACE('',(#10871),#3226,.F.);
#95845=ADVANCED_FACE('',(#10872),#91332,.F.);
#95846=ADVANCED_FACE('',(#10873),#91333,.F.);
#95847=ADVANCED_FACE('',(#10874),#3227,.F.);
#95848=ADVANCED_FACE('',(#10875),#3228,.F.);
#95849=ADVANCED_FACE('',(#10876),#91334,.F.);
#95850=ADVANCED_FACE('',(#10877),#91335,.F.);
#95851=ADVANCED_FACE('',(#10878),#3229,.F.);
#95852=ADVANCED_FACE('',(#10879),#91336,.F.);
#95853=ADVANCED_FACE('',(#10880),#6154,.F.);
#95854=ADVANCED_FACE('',(#10881),#3230,.F.);
#95855=ADVANCED_FACE('',(#10882),#3231,.F.);
#95856=ADVANCED_FACE('',(#10883),#91337,.F.);
#95857=ADVANCED_FACE('',(#10884),#91338,.F.);
#95858=ADVANCED_FACE('',(#10885),#3232,.F.);
#95859=ADVANCED_FACE('',(#10886),#3233,.F.);
#95860=ADVANCED_FACE('',(#10887),#6155,.F.);
#95861=ADVANCED_FACE('',(#10888),#91339,.F.);
#95862=ADVANCED_FACE('',(#10889),#3234,.F.);
#95863=ADVANCED_FACE('',(#10890),#91340,.F.);
#95864=ADVANCED_FACE('',(#10891),#91341,.F.);
#95865=ADVANCED_FACE('',(#10892),#3235,.F.);
#95866=ADVANCED_FACE('',(#10893),#3236,.F.);
#95867=ADVANCED_FACE('',(#10894),#91342,.F.);
#95868=ADVANCED_FACE('',(#10895),#91343,.F.);
#95869=ADVANCED_FACE('',(#10896),#3237,.F.);
#95870=ADVANCED_FACE('',(#10897),#91344,.F.);
#95871=ADVANCED_FACE('',(#10898),#7051,.F.);
#95872=ADVANCED_FACE('',(#10899),#7052,.T.);
#95873=ADVANCED_FACE('',(#10900),#7053,.F.);
#95874=ADVANCED_FACE('',(#10901),#7054,.F.);
#95875=ADVANCED_FACE('',(#10902),#7055,.T.);
#95876=ADVANCED_FACE('',(#10903),#7056,.F.);
#95877=ADVANCED_FACE('',(#10904),#7057,.F.);
#95878=ADVANCED_FACE('',(#10905),#7058,.T.);
#95879=ADVANCED_FACE('',(#10906),#7059,.F.);
#95880=ADVANCED_FACE('',(#10907),#7060,.F.);
#95881=ADVANCED_FACE('',(#10908),#7061,.T.);
#95882=ADVANCED_FACE('',(#10909),#7062,.F.);
#95883=ADVANCED_FACE('',(#10910),#7063,.F.);
#95884=ADVANCED_FACE('',(#10911),#7064,.T.);
#95885=ADVANCED_FACE('',(#10912),#7065,.F.);
#95886=ADVANCED_FACE('',(#10913),#7066,.F.);
#95887=ADVANCED_FACE('',(#10914),#7067,.T.);
#95888=ADVANCED_FACE('',(#10915),#7068,.F.);
#95889=ADVANCED_FACE('',(#10916),#7069,.F.);
#95890=ADVANCED_FACE('',(#10917),#7070,.T.);
#95891=ADVANCED_FACE('',(#10918),#7071,.F.);
#95892=ADVANCED_FACE('',(#10919),#7072,.F.);
#95893=ADVANCED_FACE('',(#10920),#7073,.T.);
#95894=ADVANCED_FACE('',(#10921),#7074,.F.);
#95895=ADVANCED_FACE('',(#10922),#7075,.F.);
#95896=ADVANCED_FACE('',(#10923),#7076,.T.);
#95897=ADVANCED_FACE('',(#10924),#7077,.F.);
#95898=ADVANCED_FACE('',(#10925),#7078,.F.);
#95899=ADVANCED_FACE('',(#10926),#7079,.T.);
#95900=ADVANCED_FACE('',(#10927),#7080,.F.);
#95901=ADVANCED_FACE('',(#10928),#7081,.F.);
#95902=ADVANCED_FACE('',(#10929),#7082,.T.);
#95903=ADVANCED_FACE('',(#10930),#7083,.F.);
#95904=ADVANCED_FACE('',(#10931),#7084,.F.);
#95905=ADVANCED_FACE('',(#10932),#7085,.T.);
#95906=ADVANCED_FACE('',(#10933),#7086,.F.);
#95907=ADVANCED_FACE('',(#10934),#7087,.F.);
#95908=ADVANCED_FACE('',(#10935),#7088,.T.);
#95909=ADVANCED_FACE('',(#10936),#7089,.F.);
#95910=ADVANCED_FACE('',(#10937),#7090,.F.);
#95911=ADVANCED_FACE('',(#10938),#7091,.T.);
#95912=ADVANCED_FACE('',(#10939),#7092,.F.);
#95913=ADVANCED_FACE('',(#10940),#7093,.F.);
#95914=ADVANCED_FACE('',(#10941),#7094,.T.);
#95915=ADVANCED_FACE('',(#10942),#7095,.F.);
#95916=ADVANCED_FACE('',(#10943),#7096,.F.);
#95917=ADVANCED_FACE('',(#10944),#7097,.T.);
#95918=ADVANCED_FACE('',(#10945),#7098,.F.);
#95919=ADVANCED_FACE('',(#10946),#7099,.F.);
#95920=ADVANCED_FACE('',(#10947),#7100,.T.);
#95921=ADVANCED_FACE('',(#10948),#7101,.F.);
#95922=ADVANCED_FACE('',(#10949),#7102,.F.);
#95923=ADVANCED_FACE('',(#10950),#7103,.T.);
#95924=ADVANCED_FACE('',(#10951),#7104,.F.);
#95925=ADVANCED_FACE('',(#10952),#7105,.F.);
#95926=ADVANCED_FACE('',(#10953),#7106,.T.);
#95927=ADVANCED_FACE('',(#10954),#7107,.F.);
#95928=ADVANCED_FACE('',(#10955),#7108,.F.);
#95929=ADVANCED_FACE('',(#10956),#7109,.T.);
#95930=ADVANCED_FACE('',(#10957),#7110,.F.);
#95931=ADVANCED_FACE('',(#10958),#7111,.F.);
#95932=ADVANCED_FACE('',(#10959),#7112,.T.);
#95933=ADVANCED_FACE('',(#10960),#7113,.F.);
#95934=ADVANCED_FACE('',(#10961),#7114,.F.);
#95935=ADVANCED_FACE('',(#10962),#7115,.T.);
#95936=ADVANCED_FACE('',(#10963),#7116,.F.);
#95937=ADVANCED_FACE('',(#10964),#7117,.F.);
#95938=ADVANCED_FACE('',(#10965),#7118,.T.);
#95939=ADVANCED_FACE('',(#10966),#7119,.F.);
#95940=ADVANCED_FACE('',(#10967),#7120,.F.);
#95941=ADVANCED_FACE('',(#10968),#7121,.T.);
#95942=ADVANCED_FACE('',(#10969),#7122,.F.);
#95943=ADVANCED_FACE('',(#10970),#7123,.F.);
#95944=ADVANCED_FACE('',(#10971),#7124,.T.);
#95945=ADVANCED_FACE('',(#10972),#7125,.F.);
#95946=ADVANCED_FACE('',(#10973),#7126,.F.);
#95947=ADVANCED_FACE('',(#10974),#7127,.T.);
#95948=ADVANCED_FACE('',(#10975),#7128,.F.);
#95949=ADVANCED_FACE('',(#10976),#7129,.F.);
#95950=ADVANCED_FACE('',(#10977),#7130,.T.);
#95951=ADVANCED_FACE('',(#10978),#7131,.F.);
#95952=ADVANCED_FACE('',(#10979),#7132,.F.);
#95953=ADVANCED_FACE('',(#10980),#7133,.T.);
#95954=ADVANCED_FACE('',(#10981),#7134,.F.);
#95955=ADVANCED_FACE('',(#10982),#7135,.F.);
#95956=ADVANCED_FACE('',(#10983),#7136,.T.);
#95957=ADVANCED_FACE('',(#10984),#7137,.F.);
#95958=ADVANCED_FACE('',(#10985),#7138,.F.);
#95959=ADVANCED_FACE('',(#10986),#7139,.T.);
#95960=ADVANCED_FACE('',(#10987),#7140,.F.);
#95961=ADVANCED_FACE('',(#10988),#7141,.F.);
#95962=ADVANCED_FACE('',(#10989),#7142,.T.);
#95963=ADVANCED_FACE('',(#10990),#7143,.F.);
#95964=ADVANCED_FACE('',(#10991),#7144,.F.);
#95965=ADVANCED_FACE('',(#10992),#7145,.T.);
#95966=ADVANCED_FACE('',(#10993),#7146,.F.);
#95967=ADVANCED_FACE('',(#10994),#7147,.F.);
#95968=ADVANCED_FACE('',(#10995),#7148,.T.);
#95969=ADVANCED_FACE('',(#10996),#7149,.F.);
#95970=ADVANCED_FACE('',(#10997),#7150,.F.);
#95971=ADVANCED_FACE('',(#10998),#7151,.T.);
#95972=ADVANCED_FACE('',(#10999),#7152,.F.);
#95973=ADVANCED_FACE('',(#11000),#7153,.F.);
#95974=ADVANCED_FACE('',(#11001),#7154,.T.);
#95975=ADVANCED_FACE('',(#11002),#7155,.F.);
#95976=ADVANCED_FACE('',(#11003),#7156,.F.);
#95977=ADVANCED_FACE('',(#11004),#7157,.T.);
#95978=ADVANCED_FACE('',(#11005),#7158,.F.);
#95979=ADVANCED_FACE('',(#11006),#7159,.F.);
#95980=ADVANCED_FACE('',(#11007),#7160,.T.);
#95981=ADVANCED_FACE('',(#11008),#7161,.F.);
#95982=ADVANCED_FACE('',(#11009),#7162,.F.);
#95983=ADVANCED_FACE('',(#11010),#7163,.T.);
#95984=ADVANCED_FACE('',(#11011),#7164,.F.);
#95985=ADVANCED_FACE('',(#11012),#7165,.F.);
#95986=ADVANCED_FACE('',(#11013),#7166,.T.);
#95987=ADVANCED_FACE('',(#11014),#7167,.F.);
#95988=ADVANCED_FACE('',(#11015),#7168,.F.);
#95989=ADVANCED_FACE('',(#11016),#7169,.T.);
#95990=ADVANCED_FACE('',(#11017),#7170,.F.);
#95991=ADVANCED_FACE('',(#11018),#7171,.F.);
#95992=ADVANCED_FACE('',(#11019),#7172,.T.);
#95993=ADVANCED_FACE('',(#11020),#7173,.F.);
#95994=ADVANCED_FACE('',(#11021),#7174,.F.);
#95995=ADVANCED_FACE('',(#11022),#7175,.T.);
#95996=ADVANCED_FACE('',(#11023),#7176,.F.);
#95997=ADVANCED_FACE('',(#11024),#7177,.F.);
#95998=ADVANCED_FACE('',(#11025),#7178,.T.);
#95999=ADVANCED_FACE('',(#11026),#7179,.F.);
#96000=ADVANCED_FACE('',(#11027),#7180,.F.);
#96001=ADVANCED_FACE('',(#11028),#7181,.T.);
#96002=ADVANCED_FACE('',(#11029),#7182,.F.);
#96003=ADVANCED_FACE('',(#11030),#7183,.F.);
#96004=ADVANCED_FACE('',(#11031),#7184,.T.);
#96005=ADVANCED_FACE('',(#11032),#7185,.F.);
#96006=ADVANCED_FACE('',(#11033),#7186,.F.);
#96007=ADVANCED_FACE('',(#11034),#7187,.T.);
#96008=ADVANCED_FACE('',(#11035),#7188,.F.);
#96009=ADVANCED_FACE('',(#11036),#7189,.F.);
#96010=ADVANCED_FACE('',(#11037),#7190,.T.);
#96011=ADVANCED_FACE('',(#11038),#7191,.F.);
#96012=ADVANCED_FACE('',(#11039),#7192,.F.);
#96013=ADVANCED_FACE('',(#11040),#7193,.T.);
#96014=ADVANCED_FACE('',(#11041),#7194,.F.);
#96015=ADVANCED_FACE('',(#11042),#7195,.F.);
#96016=ADVANCED_FACE('',(#11043),#7196,.T.);
#96017=ADVANCED_FACE('',(#11044),#7197,.F.);
#96018=ADVANCED_FACE('',(#11045),#7198,.F.);
#96019=ADVANCED_FACE('',(#11046),#7199,.T.);
#96020=ADVANCED_FACE('',(#11047),#7200,.F.);
#96021=ADVANCED_FACE('',(#11048),#7201,.F.);
#96022=ADVANCED_FACE('',(#11049),#7202,.T.);
#96023=ADVANCED_FACE('',(#11050),#7203,.F.);
#96024=ADVANCED_FACE('',(#11051),#7204,.F.);
#96025=ADVANCED_FACE('',(#11052),#7205,.T.);
#96026=ADVANCED_FACE('',(#11053),#7206,.F.);
#96027=ADVANCED_FACE('',(#11054),#7207,.F.);
#96028=ADVANCED_FACE('',(#11055),#7208,.T.);
#96029=ADVANCED_FACE('',(#11056),#7209,.F.);
#96030=ADVANCED_FACE('',(#11057),#7210,.F.);
#96031=ADVANCED_FACE('',(#11058),#7211,.T.);
#96032=ADVANCED_FACE('',(#11059),#7212,.F.);
#96033=ADVANCED_FACE('',(#11060),#7213,.F.);
#96034=ADVANCED_FACE('',(#11061),#7214,.T.);
#96035=ADVANCED_FACE('',(#11062),#7215,.F.);
#96036=ADVANCED_FACE('',(#11063),#7216,.F.);
#96037=ADVANCED_FACE('',(#11064),#7217,.T.);
#96038=ADVANCED_FACE('',(#11065),#7218,.F.);
#96039=ADVANCED_FACE('',(#11066),#7219,.F.);
#96040=ADVANCED_FACE('',(#11067),#7220,.T.);
#96041=ADVANCED_FACE('',(#11068),#7221,.F.);
#96042=ADVANCED_FACE('',(#11069),#7222,.F.);
#96043=ADVANCED_FACE('',(#11070),#7223,.T.);
#96044=ADVANCED_FACE('',(#11071),#7224,.F.);
#96045=ADVANCED_FACE('',(#11072),#7225,.F.);
#96046=ADVANCED_FACE('',(#11073),#7226,.T.);
#96047=ADVANCED_FACE('',(#11074),#7227,.F.);
#96048=ADVANCED_FACE('',(#11075),#91345,.T.);
#96049=ADVANCED_FACE('',(#11076),#91346,.T.);
#96050=ADVANCED_FACE('',(#11077),#91347,.T.);
#96051=ADVANCED_FACE('',(#11078),#91348,.T.);
#96052=ADVANCED_FACE('',(#11079),#91349,.T.);
#96053=ADVANCED_FACE('',(#11080),#91350,.T.);
#96054=ADVANCED_FACE('',(#11081),#91351,.T.);
#96055=ADVANCED_FACE('',(#11082),#91352,.T.);
#96056=ADVANCED_FACE('',(#11083),#91353,.T.);
#96057=ADVANCED_FACE('',(#11084),#91354,.T.);
#96058=ADVANCED_FACE('',(#11085),#91355,.T.);
#96059=ADVANCED_FACE('',(#11086),#91356,.T.);
#96060=ADVANCED_FACE('',(#11087),#91357,.T.);
#96061=ADVANCED_FACE('',(#11088),#91358,.T.);
#96062=ADVANCED_FACE('',(#11089),#91359,.T.);
#96063=ADVANCED_FACE('',(#11090),#91360,.T.);
#96064=ADVANCED_FACE('',(#11091),#91361,.T.);
#96065=ADVANCED_FACE('',(#11092),#91362,.T.);
#96066=ADVANCED_FACE('',(#11093),#91363,.T.);
#96067=ADVANCED_FACE('',(#11094),#91364,.T.);
#96068=ADVANCED_FACE('',(#11095),#91365,.T.);
#96069=ADVANCED_FACE('',(#11096),#91366,.T.);
#96070=ADVANCED_FACE('',(#11097),#91367,.T.);
#96071=ADVANCED_FACE('',(#11098),#91368,.T.);
#96072=ADVANCED_FACE('',(#11099),#91369,.T.);
#96073=ADVANCED_FACE('',(#11100),#91370,.T.);
#96074=ADVANCED_FACE('',(#11101),#91371,.T.);
#96075=ADVANCED_FACE('',(#11102),#91372,.T.);
#96076=ADVANCED_FACE('',(#11103),#91373,.T.);
#96077=ADVANCED_FACE('',(#11104),#91374,.T.);
#96078=ADVANCED_FACE('',(#11105),#91375,.T.);
#96079=ADVANCED_FACE('',(#11106),#91376,.T.);
#96080=ADVANCED_FACE('',(#11107),#91377,.T.);
#96081=ADVANCED_FACE('',(#11108),#91378,.T.);
#96082=ADVANCED_FACE('',(#11109),#91379,.T.);
#96083=ADVANCED_FACE('',(#11110),#91380,.T.);
#96084=ADVANCED_FACE('',(#11111),#91381,.T.);
#96085=ADVANCED_FACE('',(#11112),#91382,.T.);
#96086=ADVANCED_FACE('',(#11113),#91383,.T.);
#96087=ADVANCED_FACE('',(#11114),#91384,.T.);
#96088=ADVANCED_FACE('',(#11115),#91385,.T.);
#96089=ADVANCED_FACE('',(#11116),#91386,.T.);
#96090=ADVANCED_FACE('',(#11117),#91387,.T.);
#96091=ADVANCED_FACE('',(#11118),#91388,.T.);
#96092=ADVANCED_FACE('',(#11119),#91389,.T.);
#96093=ADVANCED_FACE('',(#11120),#91390,.T.);
#96094=ADVANCED_FACE('',(#11121),#91391,.T.);
#96095=ADVANCED_FACE('',(#11122),#91392,.T.);
#96096=ADVANCED_FACE('',(#11123),#91393,.T.);
#96097=ADVANCED_FACE('',(#11124),#91394,.T.);
#96098=ADVANCED_FACE('',(#11125),#91395,.T.);
#96099=ADVANCED_FACE('',(#11126),#91396,.T.);
#96100=ADVANCED_FACE('',(#11127),#91397,.T.);
#96101=ADVANCED_FACE('',(#11128),#91398,.T.);
#96102=ADVANCED_FACE('',(#11129),#91399,.T.);
#96103=ADVANCED_FACE('',(#11130),#91400,.T.);
#96104=ADVANCED_FACE('',(#11131),#91401,.T.);
#96105=ADVANCED_FACE('',(#11132),#91402,.T.);
#96106=ADVANCED_FACE('',(#11133),#91403,.T.);
#96107=ADVANCED_FACE('',(#11134),#91404,.T.);
#96108=ADVANCED_FACE('',(#11135),#91405,.T.);
#96109=ADVANCED_FACE('',(#11136),#91406,.T.);
#96110=ADVANCED_FACE('',(#11137),#91407,.T.);
#96111=ADVANCED_FACE('',(#11138),#91408,.T.);
#96112=ADVANCED_FACE('',(#11139),#91409,.T.);
#96113=ADVANCED_FACE('',(#11140),#91410,.T.);
#96114=ADVANCED_FACE('',(#11141),#91411,.T.);
#96115=ADVANCED_FACE('',(#11142),#91412,.T.);
#96116=ADVANCED_FACE('',(#11143),#91413,.T.);
#96117=ADVANCED_FACE('',(#11144),#91414,.T.);
#96118=ADVANCED_FACE('',(#11145),#91415,.T.);
#96119=ADVANCED_FACE('',(#11146),#91416,.T.);
#96120=ADVANCED_FACE('',(#11147),#91417,.T.);
#96121=ADVANCED_FACE('',(#11148),#91418,.T.);
#96122=ADVANCED_FACE('',(#11149),#91419,.T.);
#96123=ADVANCED_FACE('',(#11150),#91420,.T.);
#96124=ADVANCED_FACE('',(#11151),#91421,.T.);
#96125=ADVANCED_FACE('',(#11152),#91422,.T.);
#96126=ADVANCED_FACE('',(#11153),#91423,.T.);
#96127=ADVANCED_FACE('',(#11154),#91424,.T.);
#96128=ADVANCED_FACE('',(#11155),#91425,.T.);
#96129=ADVANCED_FACE('',(#11156),#91426,.T.);
#96130=ADVANCED_FACE('',(#11157),#91427,.T.);
#96131=ADVANCED_FACE('',(#11158),#91428,.T.);
#96132=ADVANCED_FACE('',(#11159),#91429,.T.);
#96133=ADVANCED_FACE('',(#11160),#91430,.T.);
#96134=ADVANCED_FACE('',(#11161),#91431,.T.);
#96135=ADVANCED_FACE('',(#11162),#91432,.T.);
#96136=ADVANCED_FACE('',(#11163),#91433,.T.);
#96137=ADVANCED_FACE('',(#11164),#91434,.T.);
#96138=ADVANCED_FACE('',(#11165),#91435,.T.);
#96139=ADVANCED_FACE('',(#11166),#91436,.T.);
#96140=ADVANCED_FACE('',(#11167),#91437,.T.);
#96141=ADVANCED_FACE('',(#11168),#91438,.T.);
#96142=ADVANCED_FACE('',(#11169),#91439,.T.);
#96143=ADVANCED_FACE('',(#11170),#91440,.T.);
#96144=ADVANCED_FACE('',(#11171),#91441,.T.);
#96145=ADVANCED_FACE('',(#11172),#91442,.T.);
#96146=ADVANCED_FACE('',(#11173),#91443,.T.);
#96147=ADVANCED_FACE('',(#11174),#91444,.T.);
#96148=ADVANCED_FACE('',(#11175),#91445,.T.);
#96149=ADVANCED_FACE('',(#11176),#91446,.T.);
#96150=ADVANCED_FACE('',(#11177),#91447,.T.);
#96151=ADVANCED_FACE('',(#11178),#91448,.T.);
#96152=ADVANCED_FACE('',(#11179),#91449,.T.);
#96153=ADVANCED_FACE('',(#11180),#91450,.T.);
#96154=ADVANCED_FACE('',(#11181),#91451,.T.);
#96155=ADVANCED_FACE('',(#11182),#91452,.T.);
#96156=ADVANCED_FACE('',(#11183),#91453,.T.);
#96157=ADVANCED_FACE('',(#11184),#91454,.T.);
#96158=ADVANCED_FACE('',(#11185),#91455,.T.);
#96159=ADVANCED_FACE('',(#11186),#91456,.T.);
#96160=ADVANCED_FACE('',(#11187),#91457,.T.);
#96161=ADVANCED_FACE('',(#11188),#91458,.T.);
#96162=ADVANCED_FACE('',(#11189),#91459,.T.);
#96163=ADVANCED_FACE('',(#11190),#91460,.T.);
#96164=ADVANCED_FACE('',(#11191),#91461,.T.);
#96165=ADVANCED_FACE('',(#11192),#91462,.T.);
#96166=ADVANCED_FACE('',(#11193),#91463,.F.);
#96167=ADVANCED_FACE('',(#11194),#3238,.F.);
#96168=ADVANCED_FACE('',(#11195),#91464,.F.);
#96169=ADVANCED_FACE('',(#11196),#91465,.F.);
#96170=ADVANCED_FACE('',(#11197),#3239,.F.);
#96171=ADVANCED_FACE('',(#11198),#3240,.F.);
#96172=ADVANCED_FACE('',(#11199),#91466,.F.);
#96173=ADVANCED_FACE('',(#11200),#91467,.F.);
#96174=ADVANCED_FACE('',(#11201),#3241,.F.);
#96175=ADVANCED_FACE('',(#11202),#91468,.F.);
#96176=ADVANCED_FACE('',(#11203),#6156,.F.);
#96177=ADVANCED_FACE('',(#11204),#3242,.F.);
#96178=ADVANCED_FACE('',(#11205),#3243,.F.);
#96179=ADVANCED_FACE('',(#11206),#91469,.F.);
#96180=ADVANCED_FACE('',(#11207),#91470,.F.);
#96181=ADVANCED_FACE('',(#11208),#3244,.F.);
#96182=ADVANCED_FACE('',(#11209),#3245,.F.);
#96183=ADVANCED_FACE('',(#11210),#6157,.F.);
#96184=ADVANCED_FACE('',(#11211),#91471,.F.);
#96185=ADVANCED_FACE('',(#11212),#3246,.F.);
#96186=ADVANCED_FACE('',(#11213),#91472,.F.);
#96187=ADVANCED_FACE('',(#11214),#91473,.F.);
#96188=ADVANCED_FACE('',(#11215),#3247,.F.);
#96189=ADVANCED_FACE('',(#11216),#3248,.F.);
#96190=ADVANCED_FACE('',(#11217),#91474,.F.);
#96191=ADVANCED_FACE('',(#11218),#91475,.F.);
#96192=ADVANCED_FACE('',(#11219),#3249,.F.);
#96193=ADVANCED_FACE('',(#11220),#91476,.F.);
#96194=ADVANCED_FACE('',(#11221),#91477,.F.);
#96195=ADVANCED_FACE('',(#11222),#3250,.F.);
#96196=ADVANCED_FACE('',(#11223),#91478,.F.);
#96197=ADVANCED_FACE('',(#11224),#91479,.F.);
#96198=ADVANCED_FACE('',(#11225),#3251,.F.);
#96199=ADVANCED_FACE('',(#11226),#3252,.F.);
#96200=ADVANCED_FACE('',(#11227),#91480,.F.);
#96201=ADVANCED_FACE('',(#11228),#91481,.F.);
#96202=ADVANCED_FACE('',(#11229),#3253,.F.);
#96203=ADVANCED_FACE('',(#11230),#91482,.F.);
#96204=ADVANCED_FACE('',(#11231),#6158,.F.);
#96205=ADVANCED_FACE('',(#11232),#3254,.F.);
#96206=ADVANCED_FACE('',(#11233),#3255,.F.);
#96207=ADVANCED_FACE('',(#11234),#91483,.F.);
#96208=ADVANCED_FACE('',(#11235),#91484,.F.);
#96209=ADVANCED_FACE('',(#11236),#3256,.F.);
#96210=ADVANCED_FACE('',(#11237),#3257,.F.);
#96211=ADVANCED_FACE('',(#11238),#6159,.F.);
#96212=ADVANCED_FACE('',(#11239),#91485,.F.);
#96213=ADVANCED_FACE('',(#11240),#3258,.F.);
#96214=ADVANCED_FACE('',(#11241),#91486,.F.);
#96215=ADVANCED_FACE('',(#11242),#91487,.F.);
#96216=ADVANCED_FACE('',(#11243),#3259,.F.);
#96217=ADVANCED_FACE('',(#11244),#3260,.F.);
#96218=ADVANCED_FACE('',(#11245),#91488,.F.);
#96219=ADVANCED_FACE('',(#11246),#91489,.F.);
#96220=ADVANCED_FACE('',(#11247),#3261,.F.);
#96221=ADVANCED_FACE('',(#11248),#91490,.F.);
#96222=ADVANCED_FACE('',(#11249),#91491,.F.);
#96223=ADVANCED_FACE('',(#11250),#3262,.F.);
#96224=ADVANCED_FACE('',(#11251),#91492,.F.);
#96225=ADVANCED_FACE('',(#11252),#91493,.F.);
#96226=ADVANCED_FACE('',(#11253),#3263,.F.);
#96227=ADVANCED_FACE('',(#11254),#3264,.F.);
#96228=ADVANCED_FACE('',(#11255),#91494,.F.);
#96229=ADVANCED_FACE('',(#11256),#91495,.F.);
#96230=ADVANCED_FACE('',(#11257),#3265,.F.);
#96231=ADVANCED_FACE('',(#11258),#91496,.F.);
#96232=ADVANCED_FACE('',(#11259),#6160,.F.);
#96233=ADVANCED_FACE('',(#11260),#3266,.F.);
#96234=ADVANCED_FACE('',(#11261),#3267,.F.);
#96235=ADVANCED_FACE('',(#11262),#91497,.F.);
#96236=ADVANCED_FACE('',(#11263),#91498,.F.);
#96237=ADVANCED_FACE('',(#11264),#3268,.F.);
#96238=ADVANCED_FACE('',(#11265),#3269,.F.);
#96239=ADVANCED_FACE('',(#11266),#6161,.F.);
#96240=ADVANCED_FACE('',(#11267),#91499,.F.);
#96241=ADVANCED_FACE('',(#11268),#3270,.F.);
#96242=ADVANCED_FACE('',(#11269),#91500,.F.);
#96243=ADVANCED_FACE('',(#11270),#91501,.F.);
#96244=ADVANCED_FACE('',(#11271),#3271,.F.);
#96245=ADVANCED_FACE('',(#11272),#3272,.F.);
#96246=ADVANCED_FACE('',(#11273),#91502,.F.);
#96247=ADVANCED_FACE('',(#11274),#91503,.F.);
#96248=ADVANCED_FACE('',(#11275),#3273,.F.);
#96249=ADVANCED_FACE('',(#11276),#91504,.F.);
#96250=ADVANCED_FACE('',(#11277),#91505,.F.);
#96251=ADVANCED_FACE('',(#11278),#3274,.F.);
#96252=ADVANCED_FACE('',(#11279),#91506,.F.);
#96253=ADVANCED_FACE('',(#11280),#91507,.F.);
#96254=ADVANCED_FACE('',(#11281),#3275,.F.);
#96255=ADVANCED_FACE('',(#11282),#3276,.F.);
#96256=ADVANCED_FACE('',(#11283),#91508,.F.);
#96257=ADVANCED_FACE('',(#11284),#91509,.F.);
#96258=ADVANCED_FACE('',(#11285),#3277,.F.);
#96259=ADVANCED_FACE('',(#11286),#91510,.F.);
#96260=ADVANCED_FACE('',(#11287),#6162,.F.);
#96261=ADVANCED_FACE('',(#11288),#3278,.F.);
#96262=ADVANCED_FACE('',(#11289),#3279,.F.);
#96263=ADVANCED_FACE('',(#11290),#91511,.F.);
#96264=ADVANCED_FACE('',(#11291),#91512,.F.);
#96265=ADVANCED_FACE('',(#11292),#3280,.F.);
#96266=ADVANCED_FACE('',(#11293),#3281,.F.);
#96267=ADVANCED_FACE('',(#11294),#6163,.F.);
#96268=ADVANCED_FACE('',(#11295),#91513,.F.);
#96269=ADVANCED_FACE('',(#11296),#3282,.F.);
#96270=ADVANCED_FACE('',(#11297),#91514,.F.);
#96271=ADVANCED_FACE('',(#11298),#91515,.F.);
#96272=ADVANCED_FACE('',(#11299),#3283,.F.);
#96273=ADVANCED_FACE('',(#11300),#3284,.F.);
#96274=ADVANCED_FACE('',(#11301),#91516,.F.);
#96275=ADVANCED_FACE('',(#11302),#91517,.F.);
#96276=ADVANCED_FACE('',(#11303),#3285,.F.);
#96277=ADVANCED_FACE('',(#11304),#91518,.F.);
#96278=ADVANCED_FACE('',(#11305),#91519,.F.);
#96279=ADVANCED_FACE('',(#11306),#3286,.F.);
#96280=ADVANCED_FACE('',(#11307),#91520,.F.);
#96281=ADVANCED_FACE('',(#11308),#91521,.F.);
#96282=ADVANCED_FACE('',(#11309),#3287,.F.);
#96283=ADVANCED_FACE('',(#11310),#3288,.F.);
#96284=ADVANCED_FACE('',(#11311),#91522,.F.);
#96285=ADVANCED_FACE('',(#11312),#91523,.F.);
#96286=ADVANCED_FACE('',(#11313),#3289,.F.);
#96287=ADVANCED_FACE('',(#11314),#91524,.F.);
#96288=ADVANCED_FACE('',(#11315),#6164,.F.);
#96289=ADVANCED_FACE('',(#11316),#3290,.F.);
#96290=ADVANCED_FACE('',(#11317),#3291,.F.);
#96291=ADVANCED_FACE('',(#11318),#91525,.F.);
#96292=ADVANCED_FACE('',(#11319),#91526,.F.);
#96293=ADVANCED_FACE('',(#11320),#3292,.F.);
#96294=ADVANCED_FACE('',(#11321),#3293,.F.);
#96295=ADVANCED_FACE('',(#11322),#6165,.F.);
#96296=ADVANCED_FACE('',(#11323),#91527,.F.);
#96297=ADVANCED_FACE('',(#11324),#3294,.F.);
#96298=ADVANCED_FACE('',(#11325),#91528,.F.);
#96299=ADVANCED_FACE('',(#11326),#91529,.F.);
#96300=ADVANCED_FACE('',(#11327),#3295,.F.);
#96301=ADVANCED_FACE('',(#11328),#3296,.F.);
#96302=ADVANCED_FACE('',(#11329),#91530,.F.);
#96303=ADVANCED_FACE('',(#11330),#91531,.F.);
#96304=ADVANCED_FACE('',(#11331),#3297,.F.);
#96305=ADVANCED_FACE('',(#11332),#91532,.F.);
#96306=ADVANCED_FACE('',(#11333),#91533,.F.);
#96307=ADVANCED_FACE('',(#11334),#3298,.F.);
#96308=ADVANCED_FACE('',(#11335),#91534,.F.);
#96309=ADVANCED_FACE('',(#11336),#91535,.F.);
#96310=ADVANCED_FACE('',(#11337),#3299,.F.);
#96311=ADVANCED_FACE('',(#11338),#3300,.F.);
#96312=ADVANCED_FACE('',(#11339),#91536,.F.);
#96313=ADVANCED_FACE('',(#11340),#91537,.F.);
#96314=ADVANCED_FACE('',(#11341),#3301,.F.);
#96315=ADVANCED_FACE('',(#11342),#91538,.F.);
#96316=ADVANCED_FACE('',(#11343),#6166,.F.);
#96317=ADVANCED_FACE('',(#11344),#3302,.F.);
#96318=ADVANCED_FACE('',(#11345),#3303,.F.);
#96319=ADVANCED_FACE('',(#11346),#91539,.F.);
#96320=ADVANCED_FACE('',(#11347),#91540,.F.);
#96321=ADVANCED_FACE('',(#11348),#3304,.F.);
#96322=ADVANCED_FACE('',(#11349),#3305,.F.);
#96323=ADVANCED_FACE('',(#11350),#6167,.F.);
#96324=ADVANCED_FACE('',(#11351),#91541,.F.);
#96325=ADVANCED_FACE('',(#11352),#3306,.F.);
#96326=ADVANCED_FACE('',(#11353),#91542,.F.);
#96327=ADVANCED_FACE('',(#11354),#91543,.F.);
#96328=ADVANCED_FACE('',(#11355),#3307,.F.);
#96329=ADVANCED_FACE('',(#11356),#3308,.F.);
#96330=ADVANCED_FACE('',(#11357),#91544,.F.);
#96331=ADVANCED_FACE('',(#11358),#91545,.F.);
#96332=ADVANCED_FACE('',(#11359),#3309,.F.);
#96333=ADVANCED_FACE('',(#11360),#91546,.F.);
#96334=ADVANCED_FACE('',(#11361),#91547,.F.);
#96335=ADVANCED_FACE('',(#11362),#3310,.F.);
#96336=ADVANCED_FACE('',(#11363),#91548,.F.);
#96337=ADVANCED_FACE('',(#11364),#91549,.F.);
#96338=ADVANCED_FACE('',(#11365),#3311,.F.);
#96339=ADVANCED_FACE('',(#11366),#3312,.F.);
#96340=ADVANCED_FACE('',(#11367),#91550,.F.);
#96341=ADVANCED_FACE('',(#11368),#91551,.F.);
#96342=ADVANCED_FACE('',(#11369),#3313,.F.);
#96343=ADVANCED_FACE('',(#11370),#91552,.F.);
#96344=ADVANCED_FACE('',(#11371),#6168,.F.);
#96345=ADVANCED_FACE('',(#11372),#3314,.F.);
#96346=ADVANCED_FACE('',(#11373),#3315,.F.);
#96347=ADVANCED_FACE('',(#11374),#91553,.F.);
#96348=ADVANCED_FACE('',(#11375),#91554,.F.);
#96349=ADVANCED_FACE('',(#11376),#3316,.F.);
#96350=ADVANCED_FACE('',(#11377),#3317,.F.);
#96351=ADVANCED_FACE('',(#11378),#6169,.F.);
#96352=ADVANCED_FACE('',(#11379),#91555,.F.);
#96353=ADVANCED_FACE('',(#11380),#3318,.F.);
#96354=ADVANCED_FACE('',(#11381),#91556,.F.);
#96355=ADVANCED_FACE('',(#11382),#91557,.F.);
#96356=ADVANCED_FACE('',(#11383),#3319,.F.);
#96357=ADVANCED_FACE('',(#11384),#3320,.F.);
#96358=ADVANCED_FACE('',(#11385),#91558,.F.);
#96359=ADVANCED_FACE('',(#11386),#91559,.F.);
#96360=ADVANCED_FACE('',(#11387),#3321,.F.);
#96361=ADVANCED_FACE('',(#11388),#91560,.F.);
#96362=ADVANCED_FACE('',(#11389),#91561,.F.);
#96363=ADVANCED_FACE('',(#11390),#3322,.F.);
#96364=ADVANCED_FACE('',(#11391),#91562,.F.);
#96365=ADVANCED_FACE('',(#11392),#91563,.F.);
#96366=ADVANCED_FACE('',(#11393),#3323,.F.);
#96367=ADVANCED_FACE('',(#11394),#3324,.F.);
#96368=ADVANCED_FACE('',(#11395),#91564,.F.);
#96369=ADVANCED_FACE('',(#11396),#91565,.F.);
#96370=ADVANCED_FACE('',(#11397),#3325,.F.);
#96371=ADVANCED_FACE('',(#11398),#91566,.F.);
#96372=ADVANCED_FACE('',(#11399),#6170,.F.);
#96373=ADVANCED_FACE('',(#11400),#3326,.F.);
#96374=ADVANCED_FACE('',(#11401),#3327,.F.);
#96375=ADVANCED_FACE('',(#11402),#91567,.F.);
#96376=ADVANCED_FACE('',(#11403),#91568,.F.);
#96377=ADVANCED_FACE('',(#11404),#3328,.F.);
#96378=ADVANCED_FACE('',(#11405),#3329,.F.);
#96379=ADVANCED_FACE('',(#11406),#6171,.F.);
#96380=ADVANCED_FACE('',(#11407),#91569,.F.);
#96381=ADVANCED_FACE('',(#11408),#3330,.F.);
#96382=ADVANCED_FACE('',(#11409),#91570,.F.);
#96383=ADVANCED_FACE('',(#11410),#91571,.F.);
#96384=ADVANCED_FACE('',(#11411),#3331,.F.);
#96385=ADVANCED_FACE('',(#11412),#3332,.F.);
#96386=ADVANCED_FACE('',(#11413),#91572,.F.);
#96387=ADVANCED_FACE('',(#11414),#91573,.F.);
#96388=ADVANCED_FACE('',(#11415),#3333,.F.);
#96389=ADVANCED_FACE('',(#11416),#91574,.F.);
#96390=ADVANCED_FACE('',(#11417),#91575,.F.);
#96391=ADVANCED_FACE('',(#11418),#3334,.F.);
#96392=ADVANCED_FACE('',(#11419),#91576,.F.);
#96393=ADVANCED_FACE('',(#11420),#91577,.F.);
#96394=ADVANCED_FACE('',(#11421),#3335,.F.);
#96395=ADVANCED_FACE('',(#11422),#3336,.F.);
#96396=ADVANCED_FACE('',(#11423),#91578,.F.);
#96397=ADVANCED_FACE('',(#11424),#91579,.F.);
#96398=ADVANCED_FACE('',(#11425),#3337,.F.);
#96399=ADVANCED_FACE('',(#11426),#91580,.F.);
#96400=ADVANCED_FACE('',(#11427),#6172,.F.);
#96401=ADVANCED_FACE('',(#11428),#3338,.F.);
#96402=ADVANCED_FACE('',(#11429),#3339,.F.);
#96403=ADVANCED_FACE('',(#11430),#91581,.F.);
#96404=ADVANCED_FACE('',(#11431),#91582,.F.);
#96405=ADVANCED_FACE('',(#11432),#3340,.F.);
#96406=ADVANCED_FACE('',(#11433),#3341,.F.);
#96407=ADVANCED_FACE('',(#11434),#6173,.F.);
#96408=ADVANCED_FACE('',(#11435),#91583,.F.);
#96409=ADVANCED_FACE('',(#11436),#3342,.F.);
#96410=ADVANCED_FACE('',(#11437),#91584,.F.);
#96411=ADVANCED_FACE('',(#11438),#91585,.F.);
#96412=ADVANCED_FACE('',(#11439),#3343,.F.);
#96413=ADVANCED_FACE('',(#11440),#3344,.F.);
#96414=ADVANCED_FACE('',(#11441),#91586,.F.);
#96415=ADVANCED_FACE('',(#11442),#91587,.F.);
#96416=ADVANCED_FACE('',(#11443),#3345,.F.);
#96417=ADVANCED_FACE('',(#11444),#91588,.F.);
#96418=ADVANCED_FACE('',(#11445),#91589,.F.);
#96419=ADVANCED_FACE('',(#11446),#3346,.F.);
#96420=ADVANCED_FACE('',(#11447),#91590,.F.);
#96421=ADVANCED_FACE('',(#11448),#91591,.F.);
#96422=ADVANCED_FACE('',(#11449),#3347,.F.);
#96423=ADVANCED_FACE('',(#11450),#3348,.F.);
#96424=ADVANCED_FACE('',(#11451),#91592,.F.);
#96425=ADVANCED_FACE('',(#11452),#91593,.F.);
#96426=ADVANCED_FACE('',(#11453),#3349,.F.);
#96427=ADVANCED_FACE('',(#11454),#91594,.F.);
#96428=ADVANCED_FACE('',(#11455),#6174,.F.);
#96429=ADVANCED_FACE('',(#11456),#3350,.F.);
#96430=ADVANCED_FACE('',(#11457),#3351,.F.);
#96431=ADVANCED_FACE('',(#11458),#91595,.F.);
#96432=ADVANCED_FACE('',(#11459),#91596,.F.);
#96433=ADVANCED_FACE('',(#11460),#3352,.F.);
#96434=ADVANCED_FACE('',(#11461),#3353,.F.);
#96435=ADVANCED_FACE('',(#11462),#6175,.F.);
#96436=ADVANCED_FACE('',(#11463),#91597,.F.);
#96437=ADVANCED_FACE('',(#11464),#3354,.F.);
#96438=ADVANCED_FACE('',(#11465),#91598,.F.);
#96439=ADVANCED_FACE('',(#11466),#91599,.F.);
#96440=ADVANCED_FACE('',(#11467),#3355,.F.);
#96441=ADVANCED_FACE('',(#11468),#3356,.F.);
#96442=ADVANCED_FACE('',(#11469),#91600,.F.);
#96443=ADVANCED_FACE('',(#11470),#91601,.F.);
#96444=ADVANCED_FACE('',(#11471),#3357,.F.);
#96445=ADVANCED_FACE('',(#11472),#91602,.F.);
#96446=ADVANCED_FACE('',(#11473),#91603,.F.);
#96447=ADVANCED_FACE('',(#11474),#3358,.F.);
#96448=ADVANCED_FACE('',(#11475),#91604,.F.);
#96449=ADVANCED_FACE('',(#11476),#91605,.F.);
#96450=ADVANCED_FACE('',(#11477),#3359,.F.);
#96451=ADVANCED_FACE('',(#11478),#3360,.F.);
#96452=ADVANCED_FACE('',(#11479),#91606,.F.);
#96453=ADVANCED_FACE('',(#11480),#91607,.F.);
#96454=ADVANCED_FACE('',(#11481),#3361,.F.);
#96455=ADVANCED_FACE('',(#11482),#91608,.F.);
#96456=ADVANCED_FACE('',(#11483),#6176,.F.);
#96457=ADVANCED_FACE('',(#11484),#3362,.F.);
#96458=ADVANCED_FACE('',(#11485),#3363,.F.);
#96459=ADVANCED_FACE('',(#11486),#91609,.F.);
#96460=ADVANCED_FACE('',(#11487),#91610,.F.);
#96461=ADVANCED_FACE('',(#11488),#3364,.F.);
#96462=ADVANCED_FACE('',(#11489),#3365,.F.);
#96463=ADVANCED_FACE('',(#11490),#6177,.F.);
#96464=ADVANCED_FACE('',(#11491),#91611,.F.);
#96465=ADVANCED_FACE('',(#11492),#3366,.F.);
#96466=ADVANCED_FACE('',(#11493),#91612,.F.);
#96467=ADVANCED_FACE('',(#11494),#91613,.F.);
#96468=ADVANCED_FACE('',(#11495),#3367,.F.);
#96469=ADVANCED_FACE('',(#11496),#3368,.F.);
#96470=ADVANCED_FACE('',(#11497),#91614,.F.);
#96471=ADVANCED_FACE('',(#11498),#91615,.F.);
#96472=ADVANCED_FACE('',(#11499),#3369,.F.);
#96473=ADVANCED_FACE('',(#11500),#91616,.F.);
#96474=ADVANCED_FACE('',(#11501),#91617,.F.);
#96475=ADVANCED_FACE('',(#11502),#3370,.F.);
#96476=ADVANCED_FACE('',(#11503),#91618,.F.);
#96477=ADVANCED_FACE('',(#11504),#91619,.F.);
#96478=ADVANCED_FACE('',(#11505),#3371,.F.);
#96479=ADVANCED_FACE('',(#11506),#3372,.F.);
#96480=ADVANCED_FACE('',(#11507),#91620,.F.);
#96481=ADVANCED_FACE('',(#11508),#91621,.F.);
#96482=ADVANCED_FACE('',(#11509),#3373,.F.);
#96483=ADVANCED_FACE('',(#11510),#91622,.F.);
#96484=ADVANCED_FACE('',(#11511),#6178,.F.);
#96485=ADVANCED_FACE('',(#11512),#3374,.F.);
#96486=ADVANCED_FACE('',(#11513),#3375,.F.);
#96487=ADVANCED_FACE('',(#11514),#91623,.F.);
#96488=ADVANCED_FACE('',(#11515),#91624,.F.);
#96489=ADVANCED_FACE('',(#11516),#3376,.F.);
#96490=ADVANCED_FACE('',(#11517),#3377,.F.);
#96491=ADVANCED_FACE('',(#11518),#6179,.F.);
#96492=ADVANCED_FACE('',(#11519),#91625,.F.);
#96493=ADVANCED_FACE('',(#11520),#3378,.F.);
#96494=ADVANCED_FACE('',(#11521),#91626,.F.);
#96495=ADVANCED_FACE('',(#11522),#91627,.F.);
#96496=ADVANCED_FACE('',(#11523),#3379,.F.);
#96497=ADVANCED_FACE('',(#11524),#3380,.F.);
#96498=ADVANCED_FACE('',(#11525),#91628,.F.);
#96499=ADVANCED_FACE('',(#11526),#91629,.F.);
#96500=ADVANCED_FACE('',(#11527),#3381,.F.);
#96501=ADVANCED_FACE('',(#11528),#91630,.F.);
#96502=ADVANCED_FACE('',(#11529),#91631,.F.);
#96503=ADVANCED_FACE('',(#11530),#3382,.F.);
#96504=ADVANCED_FACE('',(#11531),#91632,.F.);
#96505=ADVANCED_FACE('',(#11532),#91633,.F.);
#96506=ADVANCED_FACE('',(#11533),#3383,.F.);
#96507=ADVANCED_FACE('',(#11534),#3384,.F.);
#96508=ADVANCED_FACE('',(#11535),#91634,.F.);
#96509=ADVANCED_FACE('',(#11536),#91635,.F.);
#96510=ADVANCED_FACE('',(#11537),#3385,.F.);
#96511=ADVANCED_FACE('',(#11538),#91636,.F.);
#96512=ADVANCED_FACE('',(#11539),#6180,.F.);
#96513=ADVANCED_FACE('',(#11540),#3386,.F.);
#96514=ADVANCED_FACE('',(#11541),#3387,.F.);
#96515=ADVANCED_FACE('',(#11542),#91637,.F.);
#96516=ADVANCED_FACE('',(#11543),#91638,.F.);
#96517=ADVANCED_FACE('',(#11544),#3388,.F.);
#96518=ADVANCED_FACE('',(#11545),#3389,.F.);
#96519=ADVANCED_FACE('',(#11546),#6181,.F.);
#96520=ADVANCED_FACE('',(#11547),#91639,.F.);
#96521=ADVANCED_FACE('',(#11548),#3390,.F.);
#96522=ADVANCED_FACE('',(#11549),#91640,.F.);
#96523=ADVANCED_FACE('',(#11550),#91641,.F.);
#96524=ADVANCED_FACE('',(#11551),#3391,.F.);
#96525=ADVANCED_FACE('',(#11552),#3392,.F.);
#96526=ADVANCED_FACE('',(#11553),#91642,.F.);
#96527=ADVANCED_FACE('',(#11554),#91643,.F.);
#96528=ADVANCED_FACE('',(#11555),#3393,.F.);
#96529=ADVANCED_FACE('',(#11556),#91644,.F.);
#96530=ADVANCED_FACE('',(#11557),#91645,.F.);
#96531=ADVANCED_FACE('',(#11558),#3394,.F.);
#96532=ADVANCED_FACE('',(#11559),#91646,.F.);
#96533=ADVANCED_FACE('',(#11560),#91647,.F.);
#96534=ADVANCED_FACE('',(#11561),#3395,.F.);
#96535=ADVANCED_FACE('',(#11562),#3396,.F.);
#96536=ADVANCED_FACE('',(#11563),#91648,.F.);
#96537=ADVANCED_FACE('',(#11564),#91649,.F.);
#96538=ADVANCED_FACE('',(#11565),#3397,.F.);
#96539=ADVANCED_FACE('',(#11566),#91650,.F.);
#96540=ADVANCED_FACE('',(#11567),#6182,.F.);
#96541=ADVANCED_FACE('',(#11568),#3398,.F.);
#96542=ADVANCED_FACE('',(#11569),#3399,.F.);
#96543=ADVANCED_FACE('',(#11570),#91651,.F.);
#96544=ADVANCED_FACE('',(#11571),#91652,.F.);
#96545=ADVANCED_FACE('',(#11572),#3400,.F.);
#96546=ADVANCED_FACE('',(#11573),#3401,.F.);
#96547=ADVANCED_FACE('',(#11574),#6183,.F.);
#96548=ADVANCED_FACE('',(#11575),#91653,.F.);
#96549=ADVANCED_FACE('',(#11576),#3402,.F.);
#96550=ADVANCED_FACE('',(#11577),#91654,.F.);
#96551=ADVANCED_FACE('',(#11578),#91655,.F.);
#96552=ADVANCED_FACE('',(#11579),#3403,.F.);
#96553=ADVANCED_FACE('',(#11580),#3404,.F.);
#96554=ADVANCED_FACE('',(#11581),#91656,.F.);
#96555=ADVANCED_FACE('',(#11582),#91657,.F.);
#96556=ADVANCED_FACE('',(#11583),#3405,.F.);
#96557=ADVANCED_FACE('',(#11584),#91658,.F.);
#96558=ADVANCED_FACE('',(#11585),#91659,.F.);
#96559=ADVANCED_FACE('',(#11586),#3406,.F.);
#96560=ADVANCED_FACE('',(#11587),#91660,.F.);
#96561=ADVANCED_FACE('',(#11588),#91661,.F.);
#96562=ADVANCED_FACE('',(#11589),#3407,.F.);
#96563=ADVANCED_FACE('',(#11590),#3408,.F.);
#96564=ADVANCED_FACE('',(#11591),#91662,.F.);
#96565=ADVANCED_FACE('',(#11592),#91663,.F.);
#96566=ADVANCED_FACE('',(#11593),#3409,.F.);
#96567=ADVANCED_FACE('',(#11594),#91664,.F.);
#96568=ADVANCED_FACE('',(#11595),#6184,.F.);
#96569=ADVANCED_FACE('',(#11596),#3410,.F.);
#96570=ADVANCED_FACE('',(#11597),#3411,.F.);
#96571=ADVANCED_FACE('',(#11598),#91665,.F.);
#96572=ADVANCED_FACE('',(#11599),#91666,.F.);
#96573=ADVANCED_FACE('',(#11600),#3412,.F.);
#96574=ADVANCED_FACE('',(#11601),#3413,.F.);
#96575=ADVANCED_FACE('',(#11602),#6185,.F.);
#96576=ADVANCED_FACE('',(#11603),#91667,.F.);
#96577=ADVANCED_FACE('',(#11604),#3414,.F.);
#96578=ADVANCED_FACE('',(#11605),#91668,.F.);
#96579=ADVANCED_FACE('',(#11606),#91669,.F.);
#96580=ADVANCED_FACE('',(#11607),#3415,.F.);
#96581=ADVANCED_FACE('',(#11608),#3416,.F.);
#96582=ADVANCED_FACE('',(#11609),#91670,.F.);
#96583=ADVANCED_FACE('',(#11610),#91671,.F.);
#96584=ADVANCED_FACE('',(#11611),#3417,.F.);
#96585=ADVANCED_FACE('',(#11612),#91672,.F.);
#96586=ADVANCED_FACE('',(#11613),#91673,.F.);
#96587=ADVANCED_FACE('',(#11614),#3418,.F.);
#96588=ADVANCED_FACE('',(#11615),#91674,.F.);
#96589=ADVANCED_FACE('',(#11616),#91675,.F.);
#96590=ADVANCED_FACE('',(#11617),#3419,.F.);
#96591=ADVANCED_FACE('',(#11618),#3420,.F.);
#96592=ADVANCED_FACE('',(#11619),#91676,.F.);
#96593=ADVANCED_FACE('',(#11620),#91677,.F.);
#96594=ADVANCED_FACE('',(#11621),#3421,.F.);
#96595=ADVANCED_FACE('',(#11622),#91678,.F.);
#96596=ADVANCED_FACE('',(#11623),#6186,.F.);
#96597=ADVANCED_FACE('',(#11624),#3422,.F.);
#96598=ADVANCED_FACE('',(#11625),#3423,.F.);
#96599=ADVANCED_FACE('',(#11626),#91679,.F.);
#96600=ADVANCED_FACE('',(#11627),#91680,.F.);
#96601=ADVANCED_FACE('',(#11628),#3424,.F.);
#96602=ADVANCED_FACE('',(#11629),#3425,.F.);
#96603=ADVANCED_FACE('',(#11630),#6187,.F.);
#96604=ADVANCED_FACE('',(#11631),#91681,.F.);
#96605=ADVANCED_FACE('',(#11632),#3426,.F.);
#96606=ADVANCED_FACE('',(#11633),#91682,.F.);
#96607=ADVANCED_FACE('',(#11634),#91683,.F.);
#96608=ADVANCED_FACE('',(#11635),#3427,.F.);
#96609=ADVANCED_FACE('',(#11636),#3428,.F.);
#96610=ADVANCED_FACE('',(#11637),#91684,.F.);
#96611=ADVANCED_FACE('',(#11638),#91685,.F.);
#96612=ADVANCED_FACE('',(#11639),#3429,.F.);
#96613=ADVANCED_FACE('',(#11640),#91686,.F.);
#96614=ADVANCED_FACE('',(#11641),#91687,.F.);
#96615=ADVANCED_FACE('',(#11642),#3430,.F.);
#96616=ADVANCED_FACE('',(#11643),#91688,.F.);
#96617=ADVANCED_FACE('',(#11644),#91689,.F.);
#96618=ADVANCED_FACE('',(#11645),#3431,.F.);
#96619=ADVANCED_FACE('',(#11646),#3432,.F.);
#96620=ADVANCED_FACE('',(#11647),#91690,.F.);
#96621=ADVANCED_FACE('',(#11648),#91691,.F.);
#96622=ADVANCED_FACE('',(#11649),#3433,.F.);
#96623=ADVANCED_FACE('',(#11650),#91692,.F.);
#96624=ADVANCED_FACE('',(#11651),#6188,.F.);
#96625=ADVANCED_FACE('',(#11652),#3434,.F.);
#96626=ADVANCED_FACE('',(#11653),#3435,.F.);
#96627=ADVANCED_FACE('',(#11654),#91693,.F.);
#96628=ADVANCED_FACE('',(#11655),#91694,.F.);
#96629=ADVANCED_FACE('',(#11656),#3436,.F.);
#96630=ADVANCED_FACE('',(#11657),#3437,.F.);
#96631=ADVANCED_FACE('',(#11658),#6189,.F.);
#96632=ADVANCED_FACE('',(#11659),#91695,.F.);
#96633=ADVANCED_FACE('',(#11660),#3438,.F.);
#96634=ADVANCED_FACE('',(#11661),#91696,.F.);
#96635=ADVANCED_FACE('',(#11662),#91697,.F.);
#96636=ADVANCED_FACE('',(#11663),#3439,.F.);
#96637=ADVANCED_FACE('',(#11664),#3440,.F.);
#96638=ADVANCED_FACE('',(#11665),#91698,.F.);
#96639=ADVANCED_FACE('',(#11666),#91699,.F.);
#96640=ADVANCED_FACE('',(#11667),#3441,.F.);
#96641=ADVANCED_FACE('',(#11668),#91700,.F.);
#96642=ADVANCED_FACE('',(#11669),#91701,.F.);
#96643=ADVANCED_FACE('',(#11670),#3442,.F.);
#96644=ADVANCED_FACE('',(#11671),#91702,.F.);
#96645=ADVANCED_FACE('',(#11672),#91703,.F.);
#96646=ADVANCED_FACE('',(#11673),#3443,.F.);
#96647=ADVANCED_FACE('',(#11674),#3444,.F.);
#96648=ADVANCED_FACE('',(#11675),#91704,.F.);
#96649=ADVANCED_FACE('',(#11676),#91705,.F.);
#96650=ADVANCED_FACE('',(#11677),#3445,.F.);
#96651=ADVANCED_FACE('',(#11678),#91706,.F.);
#96652=ADVANCED_FACE('',(#11679),#6190,.F.);
#96653=ADVANCED_FACE('',(#11680),#3446,.F.);
#96654=ADVANCED_FACE('',(#11681),#3447,.F.);
#96655=ADVANCED_FACE('',(#11682),#91707,.F.);
#96656=ADVANCED_FACE('',(#11683),#91708,.F.);
#96657=ADVANCED_FACE('',(#11684),#3448,.F.);
#96658=ADVANCED_FACE('',(#11685),#3449,.F.);
#96659=ADVANCED_FACE('',(#11686),#6191,.F.);
#96660=ADVANCED_FACE('',(#11687),#91709,.F.);
#96661=ADVANCED_FACE('',(#11688),#3450,.F.);
#96662=ADVANCED_FACE('',(#11689),#91710,.F.);
#96663=ADVANCED_FACE('',(#11690),#91711,.F.);
#96664=ADVANCED_FACE('',(#11691),#3451,.F.);
#96665=ADVANCED_FACE('',(#11692),#3452,.F.);
#96666=ADVANCED_FACE('',(#11693),#91712,.F.);
#96667=ADVANCED_FACE('',(#11694),#91713,.F.);
#96668=ADVANCED_FACE('',(#11695),#3453,.F.);
#96669=ADVANCED_FACE('',(#11696),#91714,.F.);
#96670=ADVANCED_FACE('',(#11697),#91715,.F.);
#96671=ADVANCED_FACE('',(#11698),#3454,.F.);
#96672=ADVANCED_FACE('',(#11699),#91716,.F.);
#96673=ADVANCED_FACE('',(#11700),#91717,.F.);
#96674=ADVANCED_FACE('',(#11701),#3455,.F.);
#96675=ADVANCED_FACE('',(#11702),#3456,.F.);
#96676=ADVANCED_FACE('',(#11703),#91718,.F.);
#96677=ADVANCED_FACE('',(#11704),#91719,.F.);
#96678=ADVANCED_FACE('',(#11705),#3457,.F.);
#96679=ADVANCED_FACE('',(#11706),#91720,.F.);
#96680=ADVANCED_FACE('',(#11707),#6192,.F.);
#96681=ADVANCED_FACE('',(#11708),#3458,.F.);
#96682=ADVANCED_FACE('',(#11709),#3459,.F.);
#96683=ADVANCED_FACE('',(#11710),#91721,.F.);
#96684=ADVANCED_FACE('',(#11711),#91722,.F.);
#96685=ADVANCED_FACE('',(#11712),#3460,.F.);
#96686=ADVANCED_FACE('',(#11713),#3461,.F.);
#96687=ADVANCED_FACE('',(#11714),#6193,.F.);
#96688=ADVANCED_FACE('',(#11715),#91723,.F.);
#96689=ADVANCED_FACE('',(#11716),#3462,.F.);
#96690=ADVANCED_FACE('',(#11717),#91724,.F.);
#96691=ADVANCED_FACE('',(#11718),#91725,.F.);
#96692=ADVANCED_FACE('',(#11719),#3463,.F.);
#96693=ADVANCED_FACE('',(#11720),#3464,.F.);
#96694=ADVANCED_FACE('',(#11721),#91726,.F.);
#96695=ADVANCED_FACE('',(#11722),#91727,.F.);
#96696=ADVANCED_FACE('',(#11723),#3465,.F.);
#96697=ADVANCED_FACE('',(#11724),#91728,.F.);
#96698=ADVANCED_FACE('',(#11725),#91729,.F.);
#96699=ADVANCED_FACE('',(#11726),#3466,.F.);
#96700=ADVANCED_FACE('',(#11727),#91730,.F.);
#96701=ADVANCED_FACE('',(#11728),#91731,.F.);
#96702=ADVANCED_FACE('',(#11729),#3467,.F.);
#96703=ADVANCED_FACE('',(#11730),#3468,.F.);
#96704=ADVANCED_FACE('',(#11731),#91732,.F.);
#96705=ADVANCED_FACE('',(#11732),#91733,.F.);
#96706=ADVANCED_FACE('',(#11733),#3469,.F.);
#96707=ADVANCED_FACE('',(#11734),#91734,.F.);
#96708=ADVANCED_FACE('',(#11735),#6194,.F.);
#96709=ADVANCED_FACE('',(#11736),#3470,.F.);
#96710=ADVANCED_FACE('',(#11737),#3471,.F.);
#96711=ADVANCED_FACE('',(#11738),#91735,.F.);
#96712=ADVANCED_FACE('',(#11739),#91736,.F.);
#96713=ADVANCED_FACE('',(#11740),#3472,.F.);
#96714=ADVANCED_FACE('',(#11741),#3473,.F.);
#96715=ADVANCED_FACE('',(#11742),#6195,.F.);
#96716=ADVANCED_FACE('',(#11743),#91737,.F.);
#96717=ADVANCED_FACE('',(#11744),#3474,.F.);
#96718=ADVANCED_FACE('',(#11745),#91738,.F.);
#96719=ADVANCED_FACE('',(#11746),#91739,.F.);
#96720=ADVANCED_FACE('',(#11747),#3475,.F.);
#96721=ADVANCED_FACE('',(#11748),#3476,.F.);
#96722=ADVANCED_FACE('',(#11749),#91740,.F.);
#96723=ADVANCED_FACE('',(#11750),#91741,.F.);
#96724=ADVANCED_FACE('',(#11751),#3477,.F.);
#96725=ADVANCED_FACE('',(#11752),#91742,.F.);
#96726=ADVANCED_FACE('',(#11753),#91743,.F.);
#96727=ADVANCED_FACE('',(#11754),#3478,.F.);
#96728=ADVANCED_FACE('',(#11755),#91744,.F.);
#96729=ADVANCED_FACE('',(#11756),#91745,.F.);
#96730=ADVANCED_FACE('',(#11757),#3479,.F.);
#96731=ADVANCED_FACE('',(#11758),#3480,.F.);
#96732=ADVANCED_FACE('',(#11759),#91746,.F.);
#96733=ADVANCED_FACE('',(#11760),#91747,.F.);
#96734=ADVANCED_FACE('',(#11761),#3481,.F.);
#96735=ADVANCED_FACE('',(#11762),#91748,.F.);
#96736=ADVANCED_FACE('',(#11763),#6196,.F.);
#96737=ADVANCED_FACE('',(#11764),#3482,.F.);
#96738=ADVANCED_FACE('',(#11765),#3483,.F.);
#96739=ADVANCED_FACE('',(#11766),#91749,.F.);
#96740=ADVANCED_FACE('',(#11767),#91750,.F.);
#96741=ADVANCED_FACE('',(#11768),#3484,.F.);
#96742=ADVANCED_FACE('',(#11769),#3485,.F.);
#96743=ADVANCED_FACE('',(#11770),#6197,.F.);
#96744=ADVANCED_FACE('',(#11771),#91751,.F.);
#96745=ADVANCED_FACE('',(#11772),#3486,.F.);
#96746=ADVANCED_FACE('',(#11773),#91752,.F.);
#96747=ADVANCED_FACE('',(#11774),#91753,.F.);
#96748=ADVANCED_FACE('',(#11775),#3487,.F.);
#96749=ADVANCED_FACE('',(#11776),#3488,.F.);
#96750=ADVANCED_FACE('',(#11777),#91754,.F.);
#96751=ADVANCED_FACE('',(#11778),#91755,.F.);
#96752=ADVANCED_FACE('',(#11779),#3489,.F.);
#96753=ADVANCED_FACE('',(#11780),#91756,.F.);
#96754=ADVANCED_FACE('',(#11781),#91757,.F.);
#96755=ADVANCED_FACE('',(#11782),#3490,.F.);
#96756=ADVANCED_FACE('',(#11783),#91758,.F.);
#96757=ADVANCED_FACE('',(#11784),#91759,.F.);
#96758=ADVANCED_FACE('',(#11785),#3491,.F.);
#96759=ADVANCED_FACE('',(#11786),#3492,.F.);
#96760=ADVANCED_FACE('',(#11787),#91760,.F.);
#96761=ADVANCED_FACE('',(#11788),#91761,.F.);
#96762=ADVANCED_FACE('',(#11789),#3493,.F.);
#96763=ADVANCED_FACE('',(#11790),#91762,.F.);
#96764=ADVANCED_FACE('',(#11791),#6198,.F.);
#96765=ADVANCED_FACE('',(#11792),#3494,.F.);
#96766=ADVANCED_FACE('',(#11793),#3495,.F.);
#96767=ADVANCED_FACE('',(#11794),#91763,.F.);
#96768=ADVANCED_FACE('',(#11795),#91764,.F.);
#96769=ADVANCED_FACE('',(#11796),#3496,.F.);
#96770=ADVANCED_FACE('',(#11797),#3497,.F.);
#96771=ADVANCED_FACE('',(#11798),#6199,.F.);
#96772=ADVANCED_FACE('',(#11799),#91765,.F.);
#96773=ADVANCED_FACE('',(#11800),#3498,.F.);
#96774=ADVANCED_FACE('',(#11801),#91766,.F.);
#96775=ADVANCED_FACE('',(#11802),#91767,.F.);
#96776=ADVANCED_FACE('',(#11803),#3499,.F.);
#96777=ADVANCED_FACE('',(#11804),#3500,.F.);
#96778=ADVANCED_FACE('',(#11805),#91768,.F.);
#96779=ADVANCED_FACE('',(#11806),#91769,.F.);
#96780=ADVANCED_FACE('',(#11807),#3501,.F.);
#96781=ADVANCED_FACE('',(#11808),#91770,.F.);
#96782=ADVANCED_FACE('',(#11809),#91771,.F.);
#96783=ADVANCED_FACE('',(#11810),#3502,.F.);
#96784=ADVANCED_FACE('',(#11811),#91772,.F.);
#96785=ADVANCED_FACE('',(#11812),#91773,.F.);
#96786=ADVANCED_FACE('',(#11813),#3503,.F.);
#96787=ADVANCED_FACE('',(#11814),#3504,.F.);
#96788=ADVANCED_FACE('',(#11815),#91774,.F.);
#96789=ADVANCED_FACE('',(#11816),#91775,.F.);
#96790=ADVANCED_FACE('',(#11817),#3505,.F.);
#96791=ADVANCED_FACE('',(#11818),#91776,.F.);
#96792=ADVANCED_FACE('',(#11819),#6200,.F.);
#96793=ADVANCED_FACE('',(#11820),#3506,.F.);
#96794=ADVANCED_FACE('',(#11821),#3507,.F.);
#96795=ADVANCED_FACE('',(#11822),#91777,.F.);
#96796=ADVANCED_FACE('',(#11823),#91778,.F.);
#96797=ADVANCED_FACE('',(#11824),#3508,.F.);
#96798=ADVANCED_FACE('',(#11825),#3509,.F.);
#96799=ADVANCED_FACE('',(#11826),#6201,.F.);
#96800=ADVANCED_FACE('',(#11827),#91779,.F.);
#96801=ADVANCED_FACE('',(#11828),#3510,.F.);
#96802=ADVANCED_FACE('',(#11829),#91780,.F.);
#96803=ADVANCED_FACE('',(#11830),#91781,.F.);
#96804=ADVANCED_FACE('',(#11831),#3511,.F.);
#96805=ADVANCED_FACE('',(#11832),#3512,.F.);
#96806=ADVANCED_FACE('',(#11833),#91782,.F.);
#96807=ADVANCED_FACE('',(#11834),#91783,.F.);
#96808=ADVANCED_FACE('',(#11835),#3513,.F.);
#96809=ADVANCED_FACE('',(#11836),#91784,.F.);
#96810=ADVANCED_FACE('',(#11837),#91785,.F.);
#96811=ADVANCED_FACE('',(#11838),#3514,.F.);
#96812=ADVANCED_FACE('',(#11839),#91786,.F.);
#96813=ADVANCED_FACE('',(#11840),#91787,.F.);
#96814=ADVANCED_FACE('',(#11841),#3515,.F.);
#96815=ADVANCED_FACE('',(#11842),#3516,.F.);
#96816=ADVANCED_FACE('',(#11843),#91788,.F.);
#96817=ADVANCED_FACE('',(#11844),#91789,.F.);
#96818=ADVANCED_FACE('',(#11845),#3517,.F.);
#96819=ADVANCED_FACE('',(#11846),#91790,.F.);
#96820=ADVANCED_FACE('',(#11847),#6202,.F.);
#96821=ADVANCED_FACE('',(#11848),#3518,.F.);
#96822=ADVANCED_FACE('',(#11849),#3519,.F.);
#96823=ADVANCED_FACE('',(#11850),#91791,.F.);
#96824=ADVANCED_FACE('',(#11851),#91792,.F.);
#96825=ADVANCED_FACE('',(#11852),#3520,.F.);
#96826=ADVANCED_FACE('',(#11853),#3521,.F.);
#96827=ADVANCED_FACE('',(#11854),#6203,.F.);
#96828=ADVANCED_FACE('',(#11855),#91793,.F.);
#96829=ADVANCED_FACE('',(#11856),#3522,.F.);
#96830=ADVANCED_FACE('',(#11857),#91794,.F.);
#96831=ADVANCED_FACE('',(#11858),#91795,.F.);
#96832=ADVANCED_FACE('',(#11859),#3523,.F.);
#96833=ADVANCED_FACE('',(#11860),#3524,.F.);
#96834=ADVANCED_FACE('',(#11861),#91796,.F.);
#96835=ADVANCED_FACE('',(#11862),#91797,.F.);
#96836=ADVANCED_FACE('',(#11863),#3525,.F.);
#96837=ADVANCED_FACE('',(#11864),#91798,.F.);
#96838=ADVANCED_FACE('',(#11865),#91799,.F.);
#96839=ADVANCED_FACE('',(#11866),#3526,.F.);
#96840=ADVANCED_FACE('',(#11867),#91800,.F.);
#96841=ADVANCED_FACE('',(#11868),#91801,.F.);
#96842=ADVANCED_FACE('',(#11869),#3527,.F.);
#96843=ADVANCED_FACE('',(#11870),#3528,.F.);
#96844=ADVANCED_FACE('',(#11871),#91802,.F.);
#96845=ADVANCED_FACE('',(#11872),#91803,.F.);
#96846=ADVANCED_FACE('',(#11873),#3529,.F.);
#96847=ADVANCED_FACE('',(#11874),#91804,.F.);
#96848=ADVANCED_FACE('',(#11875),#6204,.F.);
#96849=ADVANCED_FACE('',(#11876),#3530,.F.);
#96850=ADVANCED_FACE('',(#11877),#3531,.F.);
#96851=ADVANCED_FACE('',(#11878),#91805,.F.);
#96852=ADVANCED_FACE('',(#11879),#91806,.F.);
#96853=ADVANCED_FACE('',(#11880),#3532,.F.);
#96854=ADVANCED_FACE('',(#11881),#3533,.F.);
#96855=ADVANCED_FACE('',(#11882),#6205,.F.);
#96856=ADVANCED_FACE('',(#11883),#91807,.F.);
#96857=ADVANCED_FACE('',(#11884),#3534,.F.);
#96858=ADVANCED_FACE('',(#11885),#91808,.F.);
#96859=ADVANCED_FACE('',(#11886),#91809,.F.);
#96860=ADVANCED_FACE('',(#11887),#3535,.F.);
#96861=ADVANCED_FACE('',(#11888),#3536,.F.);
#96862=ADVANCED_FACE('',(#11889),#91810,.F.);
#96863=ADVANCED_FACE('',(#11890),#91811,.F.);
#96864=ADVANCED_FACE('',(#11891),#3537,.F.);
#96865=ADVANCED_FACE('',(#11892),#91812,.F.);
#96866=ADVANCED_FACE('',(#11893),#91813,.F.);
#96867=ADVANCED_FACE('',(#11894),#3538,.F.);
#96868=ADVANCED_FACE('',(#11895),#91814,.F.);
#96869=ADVANCED_FACE('',(#11896),#91815,.F.);
#96870=ADVANCED_FACE('',(#11897),#3539,.F.);
#96871=ADVANCED_FACE('',(#11898),#3540,.F.);
#96872=ADVANCED_FACE('',(#11899),#91816,.F.);
#96873=ADVANCED_FACE('',(#11900),#91817,.F.);
#96874=ADVANCED_FACE('',(#11901),#3541,.F.);
#96875=ADVANCED_FACE('',(#11902),#91818,.F.);
#96876=ADVANCED_FACE('',(#11903),#6206,.F.);
#96877=ADVANCED_FACE('',(#11904),#3542,.F.);
#96878=ADVANCED_FACE('',(#11905),#3543,.F.);
#96879=ADVANCED_FACE('',(#11906),#91819,.F.);
#96880=ADVANCED_FACE('',(#11907),#91820,.F.);
#96881=ADVANCED_FACE('',(#11908),#3544,.F.);
#96882=ADVANCED_FACE('',(#11909),#3545,.F.);
#96883=ADVANCED_FACE('',(#11910),#6207,.F.);
#96884=ADVANCED_FACE('',(#11911),#91821,.F.);
#96885=ADVANCED_FACE('',(#11912),#3546,.F.);
#96886=ADVANCED_FACE('',(#11913),#91822,.F.);
#96887=ADVANCED_FACE('',(#11914),#91823,.F.);
#96888=ADVANCED_FACE('',(#11915),#3547,.F.);
#96889=ADVANCED_FACE('',(#11916),#3548,.F.);
#96890=ADVANCED_FACE('',(#11917),#91824,.F.);
#96891=ADVANCED_FACE('',(#11918),#91825,.F.);
#96892=ADVANCED_FACE('',(#11919),#3549,.F.);
#96893=ADVANCED_FACE('',(#11920),#91826,.F.);
#96894=ADVANCED_FACE('',(#11921),#91827,.F.);
#96895=ADVANCED_FACE('',(#11922),#3550,.F.);
#96896=ADVANCED_FACE('',(#11923),#91828,.F.);
#96897=ADVANCED_FACE('',(#11924),#91829,.F.);
#96898=ADVANCED_FACE('',(#11925),#3551,.F.);
#96899=ADVANCED_FACE('',(#11926),#3552,.F.);
#96900=ADVANCED_FACE('',(#11927),#91830,.F.);
#96901=ADVANCED_FACE('',(#11928),#91831,.F.);
#96902=ADVANCED_FACE('',(#11929),#3553,.F.);
#96903=ADVANCED_FACE('',(#11930),#91832,.F.);
#96904=ADVANCED_FACE('',(#11931),#6208,.F.);
#96905=ADVANCED_FACE('',(#11932),#3554,.F.);
#96906=ADVANCED_FACE('',(#11933),#3555,.F.);
#96907=ADVANCED_FACE('',(#11934),#91833,.F.);
#96908=ADVANCED_FACE('',(#11935),#91834,.F.);
#96909=ADVANCED_FACE('',(#11936),#3556,.F.);
#96910=ADVANCED_FACE('',(#11937),#3557,.F.);
#96911=ADVANCED_FACE('',(#11938),#6209,.F.);
#96912=ADVANCED_FACE('',(#11939),#91835,.F.);
#96913=ADVANCED_FACE('',(#11940),#3558,.F.);
#96914=ADVANCED_FACE('',(#11941),#91836,.F.);
#96915=ADVANCED_FACE('',(#11942),#91837,.F.);
#96916=ADVANCED_FACE('',(#11943),#3559,.F.);
#96917=ADVANCED_FACE('',(#11944),#3560,.F.);
#96918=ADVANCED_FACE('',(#11945),#91838,.F.);
#96919=ADVANCED_FACE('',(#11946),#91839,.F.);
#96920=ADVANCED_FACE('',(#11947),#3561,.F.);
#96921=ADVANCED_FACE('',(#11948),#91840,.F.);
#96922=ADVANCED_FACE('',(#11949),#91841,.F.);
#96923=ADVANCED_FACE('',(#11950),#3562,.F.);
#96924=ADVANCED_FACE('',(#11951),#91842,.F.);
#96925=ADVANCED_FACE('',(#11952),#91843,.F.);
#96926=ADVANCED_FACE('',(#11953),#3563,.F.);
#96927=ADVANCED_FACE('',(#11954),#3564,.F.);
#96928=ADVANCED_FACE('',(#11955),#91844,.F.);
#96929=ADVANCED_FACE('',(#11956),#91845,.F.);
#96930=ADVANCED_FACE('',(#11957),#3565,.F.);
#96931=ADVANCED_FACE('',(#11958),#91846,.F.);
#96932=ADVANCED_FACE('',(#11959),#6210,.F.);
#96933=ADVANCED_FACE('',(#11960),#3566,.F.);
#96934=ADVANCED_FACE('',(#11961),#3567,.F.);
#96935=ADVANCED_FACE('',(#11962),#91847,.F.);
#96936=ADVANCED_FACE('',(#11963),#91848,.F.);
#96937=ADVANCED_FACE('',(#11964),#3568,.F.);
#96938=ADVANCED_FACE('',(#11965),#3569,.F.);
#96939=ADVANCED_FACE('',(#11966),#6211,.F.);
#96940=ADVANCED_FACE('',(#11967),#91849,.F.);
#96941=ADVANCED_FACE('',(#11968),#3570,.F.);
#96942=ADVANCED_FACE('',(#11969),#91850,.F.);
#96943=ADVANCED_FACE('',(#11970),#91851,.F.);
#96944=ADVANCED_FACE('',(#11971),#3571,.F.);
#96945=ADVANCED_FACE('',(#11972),#3572,.F.);
#96946=ADVANCED_FACE('',(#11973),#91852,.F.);
#96947=ADVANCED_FACE('',(#11974),#91853,.F.);
#96948=ADVANCED_FACE('',(#11975),#3573,.F.);
#96949=ADVANCED_FACE('',(#11976),#91854,.F.);
#96950=ADVANCED_FACE('',(#11977),#91855,.F.);
#96951=ADVANCED_FACE('',(#11978),#3574,.F.);
#96952=ADVANCED_FACE('',(#11979),#91856,.F.);
#96953=ADVANCED_FACE('',(#11980),#91857,.F.);
#96954=ADVANCED_FACE('',(#11981),#3575,.F.);
#96955=ADVANCED_FACE('',(#11982),#3576,.F.);
#96956=ADVANCED_FACE('',(#11983),#91858,.F.);
#96957=ADVANCED_FACE('',(#11984),#91859,.F.);
#96958=ADVANCED_FACE('',(#11985),#3577,.F.);
#96959=ADVANCED_FACE('',(#11986),#91860,.F.);
#96960=ADVANCED_FACE('',(#11987),#6212,.F.);
#96961=ADVANCED_FACE('',(#11988),#3578,.F.);
#96962=ADVANCED_FACE('',(#11989),#3579,.F.);
#96963=ADVANCED_FACE('',(#11990),#91861,.F.);
#96964=ADVANCED_FACE('',(#11991),#91862,.F.);
#96965=ADVANCED_FACE('',(#11992),#3580,.F.);
#96966=ADVANCED_FACE('',(#11993),#3581,.F.);
#96967=ADVANCED_FACE('',(#11994),#6213,.F.);
#96968=ADVANCED_FACE('',(#11995),#91863,.F.);
#96969=ADVANCED_FACE('',(#11996),#3582,.F.);
#96970=ADVANCED_FACE('',(#11997),#91864,.F.);
#96971=ADVANCED_FACE('',(#11998),#91865,.F.);
#96972=ADVANCED_FACE('',(#11999),#3583,.F.);
#96973=ADVANCED_FACE('',(#12000),#3584,.F.);
#96974=ADVANCED_FACE('',(#12001),#91866,.F.);
#96975=ADVANCED_FACE('',(#12002),#91867,.F.);
#96976=ADVANCED_FACE('',(#12003),#3585,.F.);
#96977=ADVANCED_FACE('',(#12004),#91868,.F.);
#96978=ADVANCED_FACE('',(#12005),#91869,.F.);
#96979=ADVANCED_FACE('',(#12006),#3586,.F.);
#96980=ADVANCED_FACE('',(#12007),#91870,.F.);
#96981=ADVANCED_FACE('',(#12008),#91871,.F.);
#96982=ADVANCED_FACE('',(#12009),#3587,.F.);
#96983=ADVANCED_FACE('',(#12010),#3588,.F.);
#96984=ADVANCED_FACE('',(#12011),#91872,.F.);
#96985=ADVANCED_FACE('',(#12012),#91873,.F.);
#96986=ADVANCED_FACE('',(#12013),#3589,.F.);
#96987=ADVANCED_FACE('',(#12014),#91874,.F.);
#96988=ADVANCED_FACE('',(#12015),#3590,.F.);
#96989=ADVANCED_FACE('',(#12016),#3591,.F.);
#96990=ADVANCED_FACE('',(#12017),#91875,.F.);
#96991=ADVANCED_FACE('',(#12018),#91876,.F.);
#96992=ADVANCED_FACE('',(#12019),#3592,.F.);
#96993=ADVANCED_FACE('',(#12020),#3593,.F.);
#96994=ADVANCED_FACE('',(#12021),#91877,.F.);
#96995=ADVANCED_FACE('',(#12022),#3594,.F.);
#96996=ADVANCED_FACE('',(#12023),#91878,.F.);
#96997=ADVANCED_FACE('',(#12024),#91879,.F.);
#96998=ADVANCED_FACE('',(#12025),#3595,.F.);
#96999=ADVANCED_FACE('',(#12026),#3596,.F.);
#97000=ADVANCED_FACE('',(#12027),#91880,.F.);
#97001=ADVANCED_FACE('',(#12028),#91881,.F.);
#97002=ADVANCED_FACE('',(#12029),#3597,.F.);
#97003=ADVANCED_FACE('',(#12030),#91882,.F.);
#97004=ADVANCED_FACE('',(#12031),#91883,.F.);
#97005=ADVANCED_FACE('',(#12032),#3598,.F.);
#97006=ADVANCED_FACE('',(#12033),#91884,.F.);
#97007=ADVANCED_FACE('',(#12034),#91885,.F.);
#97008=ADVANCED_FACE('',(#12035),#3599,.F.);
#97009=ADVANCED_FACE('',(#12036),#3600,.F.);
#97010=ADVANCED_FACE('',(#12037),#91886,.F.);
#97011=ADVANCED_FACE('',(#12038),#91887,.F.);
#97012=ADVANCED_FACE('',(#12039),#3601,.F.);
#97013=ADVANCED_FACE('',(#12040),#91888,.F.);
#97014=ADVANCED_FACE('',(#12041),#6214,.F.);
#97015=ADVANCED_FACE('',(#12042),#3602,.F.);
#97016=ADVANCED_FACE('',(#12043),#3603,.F.);
#97017=ADVANCED_FACE('',(#12044),#91889,.F.);
#97018=ADVANCED_FACE('',(#12045),#91890,.F.);
#97019=ADVANCED_FACE('',(#12046),#3604,.F.);
#97020=ADVANCED_FACE('',(#12047),#3605,.F.);
#97021=ADVANCED_FACE('',(#12048),#6215,.F.);
#97022=ADVANCED_FACE('',(#12049),#91891,.F.);
#97023=ADVANCED_FACE('',(#12050),#3606,.F.);
#97024=ADVANCED_FACE('',(#12051),#91892,.F.);
#97025=ADVANCED_FACE('',(#12052),#91893,.F.);
#97026=ADVANCED_FACE('',(#12053),#3607,.F.);
#97027=ADVANCED_FACE('',(#12054),#3608,.F.);
#97028=ADVANCED_FACE('',(#12055),#91894,.F.);
#97029=ADVANCED_FACE('',(#12056),#91895,.F.);
#97030=ADVANCED_FACE('',(#12057),#3609,.F.);
#97031=ADVANCED_FACE('',(#12058),#91896,.F.);
#97032=ADVANCED_FACE('',(#12059),#91897,.F.);
#97033=ADVANCED_FACE('',(#12060),#3610,.F.);
#97034=ADVANCED_FACE('',(#12061),#91898,.F.);
#97035=ADVANCED_FACE('',(#12062),#91899,.F.);
#97036=ADVANCED_FACE('',(#12063),#3611,.F.);
#97037=ADVANCED_FACE('',(#12064),#3612,.F.);
#97038=ADVANCED_FACE('',(#12065),#91900,.F.);
#97039=ADVANCED_FACE('',(#12066),#91901,.F.);
#97040=ADVANCED_FACE('',(#12067),#3613,.F.);
#97041=ADVANCED_FACE('',(#12068),#91902,.F.);
#97042=ADVANCED_FACE('',(#12069),#6216,.F.);
#97043=ADVANCED_FACE('',(#12070),#3614,.F.);
#97044=ADVANCED_FACE('',(#12071),#3615,.F.);
#97045=ADVANCED_FACE('',(#12072),#91903,.F.);
#97046=ADVANCED_FACE('',(#12073),#91904,.F.);
#97047=ADVANCED_FACE('',(#12074),#3616,.F.);
#97048=ADVANCED_FACE('',(#12075),#3617,.F.);
#97049=ADVANCED_FACE('',(#12076),#6217,.F.);
#97050=ADVANCED_FACE('',(#12077),#91905,.F.);
#97051=ADVANCED_FACE('',(#12078),#3618,.F.);
#97052=ADVANCED_FACE('',(#12079),#91906,.F.);
#97053=ADVANCED_FACE('',(#12080),#91907,.F.);
#97054=ADVANCED_FACE('',(#12081),#3619,.F.);
#97055=ADVANCED_FACE('',(#12082),#3620,.F.);
#97056=ADVANCED_FACE('',(#12083),#91908,.F.);
#97057=ADVANCED_FACE('',(#12084),#91909,.F.);
#97058=ADVANCED_FACE('',(#12085),#3621,.F.);
#97059=ADVANCED_FACE('',(#12086),#91910,.F.);
#97060=ADVANCED_FACE('',(#12087),#91911,.F.);
#97061=ADVANCED_FACE('',(#12088),#3622,.F.);
#97062=ADVANCED_FACE('',(#12089),#91912,.F.);
#97063=ADVANCED_FACE('',(#12090),#91913,.F.);
#97064=ADVANCED_FACE('',(#12091),#3623,.F.);
#97065=ADVANCED_FACE('',(#12092),#3624,.F.);
#97066=ADVANCED_FACE('',(#12093),#91914,.F.);
#97067=ADVANCED_FACE('',(#12094),#91915,.F.);
#97068=ADVANCED_FACE('',(#12095),#3625,.F.);
#97069=ADVANCED_FACE('',(#12096),#91916,.F.);
#97070=ADVANCED_FACE('',(#12097),#6218,.F.);
#97071=ADVANCED_FACE('',(#12098),#3626,.F.);
#97072=ADVANCED_FACE('',(#12099),#3627,.F.);
#97073=ADVANCED_FACE('',(#12100),#91917,.F.);
#97074=ADVANCED_FACE('',(#12101),#91918,.F.);
#97075=ADVANCED_FACE('',(#12102),#3628,.F.);
#97076=ADVANCED_FACE('',(#12103),#3629,.F.);
#97077=ADVANCED_FACE('',(#12104),#6219,.F.);
#97078=ADVANCED_FACE('',(#12105),#91919,.F.);
#97079=ADVANCED_FACE('',(#12106),#3630,.F.);
#97080=ADVANCED_FACE('',(#12107),#91920,.F.);
#97081=ADVANCED_FACE('',(#12108),#91921,.F.);
#97082=ADVANCED_FACE('',(#12109),#3631,.F.);
#97083=ADVANCED_FACE('',(#12110),#3632,.F.);
#97084=ADVANCED_FACE('',(#12111),#91922,.F.);
#97085=ADVANCED_FACE('',(#12112),#91923,.F.);
#97086=ADVANCED_FACE('',(#12113),#3633,.F.);
#97087=ADVANCED_FACE('',(#12114),#91924,.F.);
#97088=ADVANCED_FACE('',(#12115),#91925,.F.);
#97089=ADVANCED_FACE('',(#12116),#3634,.F.);
#97090=ADVANCED_FACE('',(#12117),#91926,.F.);
#97091=ADVANCED_FACE('',(#12118),#91927,.F.);
#97092=ADVANCED_FACE('',(#12119),#3635,.F.);
#97093=ADVANCED_FACE('',(#12120),#3636,.F.);
#97094=ADVANCED_FACE('',(#12121),#91928,.F.);
#97095=ADVANCED_FACE('',(#12122),#91929,.F.);
#97096=ADVANCED_FACE('',(#12123),#3637,.F.);
#97097=ADVANCED_FACE('',(#12124),#91930,.F.);
#97098=ADVANCED_FACE('',(#12125),#6220,.F.);
#97099=ADVANCED_FACE('',(#12126),#3638,.F.);
#97100=ADVANCED_FACE('',(#12127),#3639,.F.);
#97101=ADVANCED_FACE('',(#12128),#91931,.F.);
#97102=ADVANCED_FACE('',(#12129),#91932,.F.);
#97103=ADVANCED_FACE('',(#12130),#3640,.F.);
#97104=ADVANCED_FACE('',(#12131),#3641,.F.);
#97105=ADVANCED_FACE('',(#12132),#6221,.F.);
#97106=ADVANCED_FACE('',(#12133),#91933,.F.);
#97107=ADVANCED_FACE('',(#12134),#3642,.F.);
#97108=ADVANCED_FACE('',(#12135),#91934,.F.);
#97109=ADVANCED_FACE('',(#12136),#91935,.F.);
#97110=ADVANCED_FACE('',(#12137),#3643,.F.);
#97111=ADVANCED_FACE('',(#12138),#3644,.F.);
#97112=ADVANCED_FACE('',(#12139),#91936,.F.);
#97113=ADVANCED_FACE('',(#12140),#91937,.F.);
#97114=ADVANCED_FACE('',(#12141),#3645,.F.);
#97115=ADVANCED_FACE('',(#12142),#91938,.F.);
#97116=ADVANCED_FACE('',(#12143),#91939,.F.);
#97117=ADVANCED_FACE('',(#12144),#3646,.F.);
#97118=ADVANCED_FACE('',(#12145),#91940,.F.);
#97119=ADVANCED_FACE('',(#12146),#91941,.F.);
#97120=ADVANCED_FACE('',(#12147),#3647,.F.);
#97121=ADVANCED_FACE('',(#12148),#3648,.F.);
#97122=ADVANCED_FACE('',(#12149),#91942,.F.);
#97123=ADVANCED_FACE('',(#12150),#91943,.F.);
#97124=ADVANCED_FACE('',(#12151),#3649,.F.);
#97125=ADVANCED_FACE('',(#12152),#91944,.F.);
#97126=ADVANCED_FACE('',(#12153),#6222,.F.);
#97127=ADVANCED_FACE('',(#12154),#3650,.F.);
#97128=ADVANCED_FACE('',(#12155),#3651,.F.);
#97129=ADVANCED_FACE('',(#12156),#91945,.F.);
#97130=ADVANCED_FACE('',(#12157),#91946,.F.);
#97131=ADVANCED_FACE('',(#12158),#3652,.F.);
#97132=ADVANCED_FACE('',(#12159),#3653,.F.);
#97133=ADVANCED_FACE('',(#12160),#6223,.F.);
#97134=ADVANCED_FACE('',(#12161),#91947,.F.);
#97135=ADVANCED_FACE('',(#12162),#3654,.F.);
#97136=ADVANCED_FACE('',(#12163),#91948,.F.);
#97137=ADVANCED_FACE('',(#12164),#91949,.F.);
#97138=ADVANCED_FACE('',(#12165),#3655,.F.);
#97139=ADVANCED_FACE('',(#12166),#3656,.F.);
#97140=ADVANCED_FACE('',(#12167),#91950,.F.);
#97141=ADVANCED_FACE('',(#12168),#91951,.F.);
#97142=ADVANCED_FACE('',(#12169),#3657,.F.);
#97143=ADVANCED_FACE('',(#12170),#91952,.F.);
#97144=ADVANCED_FACE('',(#12171),#91953,.F.);
#97145=ADVANCED_FACE('',(#12172),#3658,.F.);
#97146=ADVANCED_FACE('',(#12173),#91954,.F.);
#97147=ADVANCED_FACE('',(#12174),#91955,.F.);
#97148=ADVANCED_FACE('',(#12175),#3659,.F.);
#97149=ADVANCED_FACE('',(#12176),#3660,.F.);
#97150=ADVANCED_FACE('',(#12177),#91956,.F.);
#97151=ADVANCED_FACE('',(#12178),#91957,.F.);
#97152=ADVANCED_FACE('',(#12179),#3661,.F.);
#97153=ADVANCED_FACE('',(#12180),#91958,.F.);
#97154=ADVANCED_FACE('',(#12181),#6224,.F.);
#97155=ADVANCED_FACE('',(#12182),#3662,.F.);
#97156=ADVANCED_FACE('',(#12183),#3663,.F.);
#97157=ADVANCED_FACE('',(#12184),#91959,.F.);
#97158=ADVANCED_FACE('',(#12185),#91960,.F.);
#97159=ADVANCED_FACE('',(#12186),#3664,.F.);
#97160=ADVANCED_FACE('',(#12187),#3665,.F.);
#97161=ADVANCED_FACE('',(#12188),#6225,.F.);
#97162=ADVANCED_FACE('',(#12189),#91961,.F.);
#97163=ADVANCED_FACE('',(#12190),#3666,.F.);
#97164=ADVANCED_FACE('',(#12191),#91962,.F.);
#97165=ADVANCED_FACE('',(#12192),#91963,.F.);
#97166=ADVANCED_FACE('',(#12193),#3667,.F.);
#97167=ADVANCED_FACE('',(#12194),#3668,.F.);
#97168=ADVANCED_FACE('',(#12195),#91964,.F.);
#97169=ADVANCED_FACE('',(#12196),#91965,.F.);
#97170=ADVANCED_FACE('',(#12197),#3669,.F.);
#97171=ADVANCED_FACE('',(#12198),#91966,.F.);
#97172=ADVANCED_FACE('',(#12199),#91967,.F.);
#97173=ADVANCED_FACE('',(#12200),#3670,.F.);
#97174=ADVANCED_FACE('',(#12201),#91968,.F.);
#97175=ADVANCED_FACE('',(#12202),#91969,.F.);
#97176=ADVANCED_FACE('',(#12203),#3671,.F.);
#97177=ADVANCED_FACE('',(#12204),#3672,.F.);
#97178=ADVANCED_FACE('',(#12205),#91970,.F.);
#97179=ADVANCED_FACE('',(#12206),#91971,.F.);
#97180=ADVANCED_FACE('',(#12207),#3673,.F.);
#97181=ADVANCED_FACE('',(#12208),#91972,.F.);
#97182=ADVANCED_FACE('',(#12209),#6226,.F.);
#97183=ADVANCED_FACE('',(#12210),#3674,.F.);
#97184=ADVANCED_FACE('',(#12211),#3675,.F.);
#97185=ADVANCED_FACE('',(#12212),#91973,.F.);
#97186=ADVANCED_FACE('',(#12213),#91974,.F.);
#97187=ADVANCED_FACE('',(#12214),#3676,.F.);
#97188=ADVANCED_FACE('',(#12215),#3677,.F.);
#97189=ADVANCED_FACE('',(#12216),#6227,.F.);
#97190=ADVANCED_FACE('',(#12217),#91975,.F.);
#97191=ADVANCED_FACE('',(#12218),#3678,.F.);
#97192=ADVANCED_FACE('',(#12219),#91976,.F.);
#97193=ADVANCED_FACE('',(#12220),#91977,.F.);
#97194=ADVANCED_FACE('',(#12221),#3679,.F.);
#97195=ADVANCED_FACE('',(#12222),#3680,.F.);
#97196=ADVANCED_FACE('',(#12223),#91978,.F.);
#97197=ADVANCED_FACE('',(#12224),#91979,.F.);
#97198=ADVANCED_FACE('',(#12225),#3681,.F.);
#97199=ADVANCED_FACE('',(#12226),#91980,.F.);
#97200=ADVANCED_FACE('',(#12227),#91981,.F.);
#97201=ADVANCED_FACE('',(#12228),#3682,.F.);
#97202=ADVANCED_FACE('',(#12229),#91982,.F.);
#97203=ADVANCED_FACE('',(#12230),#91983,.F.);
#97204=ADVANCED_FACE('',(#12231),#3683,.F.);
#97205=ADVANCED_FACE('',(#12232),#3684,.F.);
#97206=ADVANCED_FACE('',(#12233),#91984,.F.);
#97207=ADVANCED_FACE('',(#12234),#91985,.F.);
#97208=ADVANCED_FACE('',(#12235),#3685,.F.);
#97209=ADVANCED_FACE('',(#12236),#91986,.F.);
#97210=ADVANCED_FACE('',(#12237),#6228,.F.);
#97211=ADVANCED_FACE('',(#12238),#3686,.F.);
#97212=ADVANCED_FACE('',(#12239),#3687,.F.);
#97213=ADVANCED_FACE('',(#12240),#91987,.F.);
#97214=ADVANCED_FACE('',(#12241),#91988,.F.);
#97215=ADVANCED_FACE('',(#12242),#3688,.F.);
#97216=ADVANCED_FACE('',(#12243),#3689,.F.);
#97217=ADVANCED_FACE('',(#12244),#6229,.F.);
#97218=ADVANCED_FACE('',(#12245),#91989,.F.);
#97219=ADVANCED_FACE('',(#12246),#3690,.F.);
#97220=ADVANCED_FACE('',(#12247),#91990,.F.);
#97221=ADVANCED_FACE('',(#12248),#91991,.F.);
#97222=ADVANCED_FACE('',(#12249),#3691,.F.);
#97223=ADVANCED_FACE('',(#12250),#3692,.F.);
#97224=ADVANCED_FACE('',(#12251),#91992,.F.);
#97225=ADVANCED_FACE('',(#12252),#91993,.F.);
#97226=ADVANCED_FACE('',(#12253),#3693,.F.);
#97227=ADVANCED_FACE('',(#12254),#91994,.F.);
#97228=ADVANCED_FACE('',(#12255),#91995,.F.);
#97229=ADVANCED_FACE('',(#12256),#3694,.F.);
#97230=ADVANCED_FACE('',(#12257),#91996,.F.);
#97231=ADVANCED_FACE('',(#12258),#91997,.F.);
#97232=ADVANCED_FACE('',(#12259),#3695,.F.);
#97233=ADVANCED_FACE('',(#12260),#3696,.F.);
#97234=ADVANCED_FACE('',(#12261),#91998,.F.);
#97235=ADVANCED_FACE('',(#12262),#91999,.F.);
#97236=ADVANCED_FACE('',(#12263),#3697,.F.);
#97237=ADVANCED_FACE('',(#12264),#92000,.F.);
#97238=ADVANCED_FACE('',(#12265),#6230,.F.);
#97239=ADVANCED_FACE('',(#12266),#3698,.F.);
#97240=ADVANCED_FACE('',(#12267),#3699,.F.);
#97241=ADVANCED_FACE('',(#12268),#92001,.F.);
#97242=ADVANCED_FACE('',(#12269),#92002,.F.);
#97243=ADVANCED_FACE('',(#12270),#3700,.F.);
#97244=ADVANCED_FACE('',(#12271),#3701,.F.);
#97245=ADVANCED_FACE('',(#12272),#6231,.F.);
#97246=ADVANCED_FACE('',(#12273),#92003,.F.);
#97247=ADVANCED_FACE('',(#12274),#3702,.F.);
#97248=ADVANCED_FACE('',(#12275),#92004,.F.);
#97249=ADVANCED_FACE('',(#12276),#92005,.F.);
#97250=ADVANCED_FACE('',(#12277),#3703,.F.);
#97251=ADVANCED_FACE('',(#12278),#3704,.F.);
#97252=ADVANCED_FACE('',(#12279),#92006,.F.);
#97253=ADVANCED_FACE('',(#12280),#92007,.F.);
#97254=ADVANCED_FACE('',(#12281),#3705,.F.);
#97255=ADVANCED_FACE('',(#12282),#92008,.F.);
#97256=ADVANCED_FACE('',(#12283),#92009,.F.);
#97257=ADVANCED_FACE('',(#12284),#3706,.F.);
#97258=ADVANCED_FACE('',(#12285),#92010,.F.);
#97259=ADVANCED_FACE('',(#12286),#92011,.F.);
#97260=ADVANCED_FACE('',(#12287),#3707,.F.);
#97261=ADVANCED_FACE('',(#12288),#3708,.F.);
#97262=ADVANCED_FACE('',(#12289),#92012,.F.);
#97263=ADVANCED_FACE('',(#12290),#92013,.F.);
#97264=ADVANCED_FACE('',(#12291),#3709,.F.);
#97265=ADVANCED_FACE('',(#12292),#92014,.F.);
#97266=ADVANCED_FACE('',(#12293),#6232,.F.);
#97267=ADVANCED_FACE('',(#12294),#3710,.F.);
#97268=ADVANCED_FACE('',(#12295),#3711,.F.);
#97269=ADVANCED_FACE('',(#12296),#92015,.F.);
#97270=ADVANCED_FACE('',(#12297),#92016,.F.);
#97271=ADVANCED_FACE('',(#12298),#3712,.F.);
#97272=ADVANCED_FACE('',(#12299),#3713,.F.);
#97273=ADVANCED_FACE('',(#12300),#6233,.F.);
#97274=ADVANCED_FACE('',(#12301),#92017,.F.);
#97275=ADVANCED_FACE('',(#12302),#3714,.F.);
#97276=ADVANCED_FACE('',(#12303),#92018,.F.);
#97277=ADVANCED_FACE('',(#12304),#92019,.F.);
#97278=ADVANCED_FACE('',(#12305),#3715,.F.);
#97279=ADVANCED_FACE('',(#12306),#3716,.F.);
#97280=ADVANCED_FACE('',(#12307),#92020,.F.);
#97281=ADVANCED_FACE('',(#12308),#92021,.F.);
#97282=ADVANCED_FACE('',(#12309),#3717,.F.);
#97283=ADVANCED_FACE('',(#12310),#92022,.F.);
#97284=ADVANCED_FACE('',(#12311),#92023,.F.);
#97285=ADVANCED_FACE('',(#12312),#3718,.F.);
#97286=ADVANCED_FACE('',(#12313),#92024,.F.);
#97287=ADVANCED_FACE('',(#12314),#92025,.F.);
#97288=ADVANCED_FACE('',(#12315),#3719,.F.);
#97289=ADVANCED_FACE('',(#12316),#3720,.F.);
#97290=ADVANCED_FACE('',(#12317),#92026,.F.);
#97291=ADVANCED_FACE('',(#12318),#92027,.F.);
#97292=ADVANCED_FACE('',(#12319),#3721,.F.);
#97293=ADVANCED_FACE('',(#12320),#92028,.F.);
#97294=ADVANCED_FACE('',(#12321),#6234,.F.);
#97295=ADVANCED_FACE('',(#12322),#3722,.F.);
#97296=ADVANCED_FACE('',(#12323),#3723,.F.);
#97297=ADVANCED_FACE('',(#12324),#92029,.F.);
#97298=ADVANCED_FACE('',(#12325),#92030,.F.);
#97299=ADVANCED_FACE('',(#12326),#3724,.F.);
#97300=ADVANCED_FACE('',(#12327),#3725,.F.);
#97301=ADVANCED_FACE('',(#12328),#6235,.F.);
#97302=ADVANCED_FACE('',(#12329),#92031,.F.);
#97303=ADVANCED_FACE('',(#12330),#3726,.F.);
#97304=ADVANCED_FACE('',(#12331),#92032,.F.);
#97305=ADVANCED_FACE('',(#12332),#92033,.F.);
#97306=ADVANCED_FACE('',(#12333),#3727,.F.);
#97307=ADVANCED_FACE('',(#12334),#3728,.F.);
#97308=ADVANCED_FACE('',(#12335),#92034,.F.);
#97309=ADVANCED_FACE('',(#12336),#92035,.F.);
#97310=ADVANCED_FACE('',(#12337),#3729,.F.);
#97311=ADVANCED_FACE('',(#12338),#92036,.F.);
#97312=ADVANCED_FACE('',(#12339),#92037,.F.);
#97313=ADVANCED_FACE('',(#12340),#3730,.F.);
#97314=ADVANCED_FACE('',(#12341),#92038,.F.);
#97315=ADVANCED_FACE('',(#12342),#92039,.F.);
#97316=ADVANCED_FACE('',(#12343),#3731,.F.);
#97317=ADVANCED_FACE('',(#12344),#3732,.F.);
#97318=ADVANCED_FACE('',(#12345),#92040,.F.);
#97319=ADVANCED_FACE('',(#12346),#92041,.F.);
#97320=ADVANCED_FACE('',(#12347),#3733,.F.);
#97321=ADVANCED_FACE('',(#12348),#92042,.F.);
#97322=ADVANCED_FACE('',(#12349),#6236,.F.);
#97323=ADVANCED_FACE('',(#12350),#3734,.F.);
#97324=ADVANCED_FACE('',(#12351),#3735,.F.);
#97325=ADVANCED_FACE('',(#12352),#92043,.F.);
#97326=ADVANCED_FACE('',(#12353),#92044,.F.);
#97327=ADVANCED_FACE('',(#12354),#3736,.F.);
#97328=ADVANCED_FACE('',(#12355),#3737,.F.);
#97329=ADVANCED_FACE('',(#12356),#6237,.F.);
#97330=ADVANCED_FACE('',(#12357),#92045,.F.);
#97331=ADVANCED_FACE('',(#12358),#3738,.F.);
#97332=ADVANCED_FACE('',(#12359),#92046,.F.);
#97333=ADVANCED_FACE('',(#12360),#92047,.F.);
#97334=ADVANCED_FACE('',(#12361),#3739,.F.);
#97335=ADVANCED_FACE('',(#12362),#3740,.F.);
#97336=ADVANCED_FACE('',(#12363),#92048,.F.);
#97337=ADVANCED_FACE('',(#12364),#92049,.F.);
#97338=ADVANCED_FACE('',(#12365),#3741,.F.);
#97339=ADVANCED_FACE('',(#12366),#92050,.F.);
#97340=ADVANCED_FACE('',(#12367),#92051,.F.);
#97341=ADVANCED_FACE('',(#12368),#3742,.F.);
#97342=ADVANCED_FACE('',(#12369),#92052,.F.);
#97343=ADVANCED_FACE('',(#12370),#92053,.F.);
#97344=ADVANCED_FACE('',(#12371),#3743,.F.);
#97345=ADVANCED_FACE('',(#12372),#3744,.F.);
#97346=ADVANCED_FACE('',(#12373),#92054,.F.);
#97347=ADVANCED_FACE('',(#12374),#92055,.F.);
#97348=ADVANCED_FACE('',(#12375),#3745,.F.);
#97349=ADVANCED_FACE('',(#12376),#92056,.F.);
#97350=ADVANCED_FACE('',(#12377),#6238,.F.);
#97351=ADVANCED_FACE('',(#12378),#3746,.F.);
#97352=ADVANCED_FACE('',(#12379),#3747,.F.);
#97353=ADVANCED_FACE('',(#12380),#92057,.F.);
#97354=ADVANCED_FACE('',(#12381),#92058,.F.);
#97355=ADVANCED_FACE('',(#12382),#3748,.F.);
#97356=ADVANCED_FACE('',(#12383),#3749,.F.);
#97357=ADVANCED_FACE('',(#12384),#6239,.F.);
#97358=ADVANCED_FACE('',(#12385),#92059,.F.);
#97359=ADVANCED_FACE('',(#12386),#3750,.F.);
#97360=ADVANCED_FACE('',(#12387),#92060,.F.);
#97361=ADVANCED_FACE('',(#12388),#92061,.F.);
#97362=ADVANCED_FACE('',(#12389),#3751,.F.);
#97363=ADVANCED_FACE('',(#12390),#3752,.F.);
#97364=ADVANCED_FACE('',(#12391),#92062,.F.);
#97365=ADVANCED_FACE('',(#12392),#92063,.F.);
#97366=ADVANCED_FACE('',(#12393),#3753,.F.);
#97367=ADVANCED_FACE('',(#12394),#92064,.F.);
#97368=ADVANCED_FACE('',(#12395),#92065,.F.);
#97369=ADVANCED_FACE('',(#12396),#3754,.F.);
#97370=ADVANCED_FACE('',(#12397),#92066,.F.);
#97371=ADVANCED_FACE('',(#12398),#92067,.F.);
#97372=ADVANCED_FACE('',(#12399),#3755,.F.);
#97373=ADVANCED_FACE('',(#12400),#3756,.F.);
#97374=ADVANCED_FACE('',(#12401),#92068,.F.);
#97375=ADVANCED_FACE('',(#12402),#92069,.F.);
#97376=ADVANCED_FACE('',(#12403),#3757,.F.);
#97377=ADVANCED_FACE('',(#12404),#92070,.F.);
#97378=ADVANCED_FACE('',(#12405),#6240,.F.);
#97379=ADVANCED_FACE('',(#12406),#3758,.F.);
#97380=ADVANCED_FACE('',(#12407),#3759,.F.);
#97381=ADVANCED_FACE('',(#12408),#92071,.F.);
#97382=ADVANCED_FACE('',(#12409),#92072,.F.);
#97383=ADVANCED_FACE('',(#12410),#3760,.F.);
#97384=ADVANCED_FACE('',(#12411),#3761,.F.);
#97385=ADVANCED_FACE('',(#12412),#6241,.F.);
#97386=ADVANCED_FACE('',(#12413),#92073,.F.);
#97387=ADVANCED_FACE('',(#12414),#3762,.F.);
#97388=ADVANCED_FACE('',(#12415),#92074,.F.);
#97389=ADVANCED_FACE('',(#12416),#92075,.F.);
#97390=ADVANCED_FACE('',(#12417),#3763,.F.);
#97391=ADVANCED_FACE('',(#12418),#3764,.F.);
#97392=ADVANCED_FACE('',(#12419),#92076,.F.);
#97393=ADVANCED_FACE('',(#12420),#92077,.F.);
#97394=ADVANCED_FACE('',(#12421),#3765,.F.);
#97395=ADVANCED_FACE('',(#12422),#92078,.F.);
#97396=ADVANCED_FACE('',(#12423),#92079,.F.);
#97397=ADVANCED_FACE('',(#12424),#3766,.F.);
#97398=ADVANCED_FACE('',(#12425),#92080,.F.);
#97399=ADVANCED_FACE('',(#12426),#92081,.F.);
#97400=ADVANCED_FACE('',(#12427),#3767,.F.);
#97401=ADVANCED_FACE('',(#12428),#3768,.F.);
#97402=ADVANCED_FACE('',(#12429),#92082,.F.);
#97403=ADVANCED_FACE('',(#12430),#92083,.F.);
#97404=ADVANCED_FACE('',(#12431),#3769,.F.);
#97405=ADVANCED_FACE('',(#12432),#92084,.F.);
#97406=ADVANCED_FACE('',(#12433),#3770,.F.);
#97407=ADVANCED_FACE('',(#12434),#3771,.F.);
#97408=ADVANCED_FACE('',(#12435),#92085,.F.);
#97409=ADVANCED_FACE('',(#12436),#92086,.F.);
#97410=ADVANCED_FACE('',(#12437),#3772,.F.);
#97411=ADVANCED_FACE('',(#12438),#3773,.F.);
#97412=ADVANCED_FACE('',(#12439),#92087,.F.);
#97413=ADVANCED_FACE('',(#12440),#3774,.F.);
#97414=ADVANCED_FACE('',(#12441),#92088,.F.);
#97415=ADVANCED_FACE('',(#12442),#92089,.F.);
#97416=ADVANCED_FACE('',(#12443),#3775,.F.);
#97417=ADVANCED_FACE('',(#12444),#3776,.F.);
#97418=ADVANCED_FACE('',(#12445),#92090,.F.);
#97419=ADVANCED_FACE('',(#12446),#92091,.F.);
#97420=ADVANCED_FACE('',(#12447),#3777,.F.);
#97421=ADVANCED_FACE('',(#12448),#92092,.F.);
#97422=ADVANCED_FACE('',(#12449),#92093,.F.);
#97423=ADVANCED_FACE('',(#12450),#3778,.F.);
#97424=ADVANCED_FACE('',(#12451),#92094,.F.);
#97425=ADVANCED_FACE('',(#12452),#92095,.F.);
#97426=ADVANCED_FACE('',(#12453),#3779,.F.);
#97427=ADVANCED_FACE('',(#12454),#3780,.F.);
#97428=ADVANCED_FACE('',(#12455),#92096,.F.);
#97429=ADVANCED_FACE('',(#12456),#92097,.F.);
#97430=ADVANCED_FACE('',(#12457),#3781,.F.);
#97431=ADVANCED_FACE('',(#12458),#92098,.F.);
#97432=ADVANCED_FACE('',(#12459),#6242,.F.);
#97433=ADVANCED_FACE('',(#12460),#3782,.F.);
#97434=ADVANCED_FACE('',(#12461),#3783,.F.);
#97435=ADVANCED_FACE('',(#12462),#92099,.F.);
#97436=ADVANCED_FACE('',(#12463),#92100,.F.);
#97437=ADVANCED_FACE('',(#12464),#3784,.F.);
#97438=ADVANCED_FACE('',(#12465),#3785,.F.);
#97439=ADVANCED_FACE('',(#12466),#6243,.F.);
#97440=ADVANCED_FACE('',(#12467),#92101,.F.);
#97441=ADVANCED_FACE('',(#12468),#3786,.F.);
#97442=ADVANCED_FACE('',(#12469),#92102,.F.);
#97443=ADVANCED_FACE('',(#12470),#92103,.F.);
#97444=ADVANCED_FACE('',(#12471),#3787,.F.);
#97445=ADVANCED_FACE('',(#12472),#3788,.F.);
#97446=ADVANCED_FACE('',(#12473),#92104,.F.);
#97447=ADVANCED_FACE('',(#12474),#92105,.F.);
#97448=ADVANCED_FACE('',(#12475),#3789,.F.);
#97449=ADVANCED_FACE('',(#12476),#92106,.F.);
#97450=ADVANCED_FACE('',(#12477),#92107,.F.);
#97451=ADVANCED_FACE('',(#12478),#3790,.F.);
#97452=ADVANCED_FACE('',(#12479),#92108,.F.);
#97453=ADVANCED_FACE('',(#12480),#92109,.F.);
#97454=ADVANCED_FACE('',(#12481),#3791,.F.);
#97455=ADVANCED_FACE('',(#12482),#3792,.F.);
#97456=ADVANCED_FACE('',(#12483),#92110,.F.);
#97457=ADVANCED_FACE('',(#12484),#92111,.F.);
#97458=ADVANCED_FACE('',(#12485),#3793,.F.);
#97459=ADVANCED_FACE('',(#12486),#92112,.F.);
#97460=ADVANCED_FACE('',(#12487),#6244,.F.);
#97461=ADVANCED_FACE('',(#12488),#3794,.F.);
#97462=ADVANCED_FACE('',(#12489),#3795,.F.);
#97463=ADVANCED_FACE('',(#12490),#92113,.F.);
#97464=ADVANCED_FACE('',(#12491),#92114,.F.);
#97465=ADVANCED_FACE('',(#12492),#3796,.F.);
#97466=ADVANCED_FACE('',(#12493),#3797,.F.);
#97467=ADVANCED_FACE('',(#12494),#6245,.F.);
#97468=ADVANCED_FACE('',(#12495),#92115,.F.);
#97469=ADVANCED_FACE('',(#12496),#3798,.F.);
#97470=ADVANCED_FACE('',(#12497),#92116,.F.);
#97471=ADVANCED_FACE('',(#12498),#92117,.F.);
#97472=ADVANCED_FACE('',(#12499),#3799,.F.);
#97473=ADVANCED_FACE('',(#12500),#3800,.F.);
#97474=ADVANCED_FACE('',(#12501),#92118,.F.);
#97475=ADVANCED_FACE('',(#12502),#92119,.F.);
#97476=ADVANCED_FACE('',(#12503),#3801,.F.);
#97477=ADVANCED_FACE('',(#12504),#92120,.F.);
#97478=ADVANCED_FACE('',(#12505),#92121,.F.);
#97479=ADVANCED_FACE('',(#12506),#3802,.F.);
#97480=ADVANCED_FACE('',(#12507),#92122,.F.);
#97481=ADVANCED_FACE('',(#12508),#92123,.F.);
#97482=ADVANCED_FACE('',(#12509),#3803,.F.);
#97483=ADVANCED_FACE('',(#12510),#3804,.F.);
#97484=ADVANCED_FACE('',(#12511),#92124,.F.);
#97485=ADVANCED_FACE('',(#12512),#92125,.F.);
#97486=ADVANCED_FACE('',(#12513),#3805,.F.);
#97487=ADVANCED_FACE('',(#12514),#92126,.F.);
#97488=ADVANCED_FACE('',(#12515),#6246,.F.);
#97489=ADVANCED_FACE('',(#12516),#3806,.F.);
#97490=ADVANCED_FACE('',(#12517),#3807,.F.);
#97491=ADVANCED_FACE('',(#12518),#92127,.F.);
#97492=ADVANCED_FACE('',(#12519),#92128,.F.);
#97493=ADVANCED_FACE('',(#12520),#3808,.F.);
#97494=ADVANCED_FACE('',(#12521),#3809,.F.);
#97495=ADVANCED_FACE('',(#12522),#6247,.F.);
#97496=ADVANCED_FACE('',(#12523),#92129,.F.);
#97497=ADVANCED_FACE('',(#12524),#3810,.F.);
#97498=ADVANCED_FACE('',(#12525),#92130,.F.);
#97499=ADVANCED_FACE('',(#12526),#92131,.F.);
#97500=ADVANCED_FACE('',(#12527),#3811,.F.);
#97501=ADVANCED_FACE('',(#12528),#3812,.F.);
#97502=ADVANCED_FACE('',(#12529),#92132,.F.);
#97503=ADVANCED_FACE('',(#12530),#92133,.F.);
#97504=ADVANCED_FACE('',(#12531),#3813,.F.);
#97505=ADVANCED_FACE('',(#12532),#92134,.F.);
#97506=ADVANCED_FACE('',(#12533),#92135,.F.);
#97507=ADVANCED_FACE('',(#12534),#3814,.F.);
#97508=ADVANCED_FACE('',(#12535),#92136,.F.);
#97509=ADVANCED_FACE('',(#12536),#92137,.F.);
#97510=ADVANCED_FACE('',(#12537),#3815,.F.);
#97511=ADVANCED_FACE('',(#12538),#3816,.F.);
#97512=ADVANCED_FACE('',(#12539),#92138,.F.);
#97513=ADVANCED_FACE('',(#12540),#92139,.F.);
#97514=ADVANCED_FACE('',(#12541),#3817,.F.);
#97515=ADVANCED_FACE('',(#12542),#92140,.F.);
#97516=ADVANCED_FACE('',(#12543),#6248,.F.);
#97517=ADVANCED_FACE('',(#12544),#3818,.F.);
#97518=ADVANCED_FACE('',(#12545),#3819,.F.);
#97519=ADVANCED_FACE('',(#12546),#92141,.F.);
#97520=ADVANCED_FACE('',(#12547),#92142,.F.);
#97521=ADVANCED_FACE('',(#12548),#3820,.F.);
#97522=ADVANCED_FACE('',(#12549),#3821,.F.);
#97523=ADVANCED_FACE('',(#12550),#6249,.F.);
#97524=ADVANCED_FACE('',(#12551),#92143,.F.);
#97525=ADVANCED_FACE('',(#12552),#3822,.F.);
#97526=ADVANCED_FACE('',(#12553),#92144,.F.);
#97527=ADVANCED_FACE('',(#12554),#92145,.F.);
#97528=ADVANCED_FACE('',(#12555),#3823,.F.);
#97529=ADVANCED_FACE('',(#12556),#3824,.F.);
#97530=ADVANCED_FACE('',(#12557),#92146,.F.);
#97531=ADVANCED_FACE('',(#12558),#92147,.F.);
#97532=ADVANCED_FACE('',(#12559),#3825,.F.);
#97533=ADVANCED_FACE('',(#12560),#92148,.F.);
#97534=ADVANCED_FACE('',(#12561),#92149,.F.);
#97535=ADVANCED_FACE('',(#12562),#3826,.F.);
#97536=ADVANCED_FACE('',(#12563),#92150,.F.);
#97537=ADVANCED_FACE('',(#12564),#92151,.F.);
#97538=ADVANCED_FACE('',(#12565),#3827,.F.);
#97539=ADVANCED_FACE('',(#12566),#3828,.F.);
#97540=ADVANCED_FACE('',(#12567),#92152,.F.);
#97541=ADVANCED_FACE('',(#12568),#92153,.F.);
#97542=ADVANCED_FACE('',(#12569),#3829,.F.);
#97543=ADVANCED_FACE('',(#12570),#92154,.F.);
#97544=ADVANCED_FACE('',(#12571),#6250,.F.);
#97545=ADVANCED_FACE('',(#12572),#3830,.F.);
#97546=ADVANCED_FACE('',(#12573),#3831,.F.);
#97547=ADVANCED_FACE('',(#12574),#92155,.F.);
#97548=ADVANCED_FACE('',(#12575),#92156,.F.);
#97549=ADVANCED_FACE('',(#12576),#3832,.F.);
#97550=ADVANCED_FACE('',(#12577),#3833,.F.);
#97551=ADVANCED_FACE('',(#12578),#6251,.F.);
#97552=ADVANCED_FACE('',(#12579),#92157,.F.);
#97553=ADVANCED_FACE('',(#12580),#3834,.F.);
#97554=ADVANCED_FACE('',(#12581),#92158,.F.);
#97555=ADVANCED_FACE('',(#12582),#92159,.F.);
#97556=ADVANCED_FACE('',(#12583),#3835,.F.);
#97557=ADVANCED_FACE('',(#12584),#3836,.F.);
#97558=ADVANCED_FACE('',(#12585),#92160,.F.);
#97559=ADVANCED_FACE('',(#12586),#92161,.F.);
#97560=ADVANCED_FACE('',(#12587),#3837,.F.);
#97561=ADVANCED_FACE('',(#12588),#92162,.F.);
#97562=ADVANCED_FACE('',(#12589),#92163,.F.);
#97563=ADVANCED_FACE('',(#12590),#3838,.F.);
#97564=ADVANCED_FACE('',(#12591),#92164,.F.);
#97565=ADVANCED_FACE('',(#12592),#92165,.F.);
#97566=ADVANCED_FACE('',(#12593),#3839,.F.);
#97567=ADVANCED_FACE('',(#12594),#3840,.F.);
#97568=ADVANCED_FACE('',(#12595),#92166,.F.);
#97569=ADVANCED_FACE('',(#12596),#92167,.F.);
#97570=ADVANCED_FACE('',(#12597),#3841,.F.);
#97571=ADVANCED_FACE('',(#12598),#92168,.F.);
#97572=ADVANCED_FACE('',(#12599),#6252,.F.);
#97573=ADVANCED_FACE('',(#12600),#3842,.F.);
#97574=ADVANCED_FACE('',(#12601),#3843,.F.);
#97575=ADVANCED_FACE('',(#12602),#92169,.F.);
#97576=ADVANCED_FACE('',(#12603),#92170,.F.);
#97577=ADVANCED_FACE('',(#12604),#3844,.F.);
#97578=ADVANCED_FACE('',(#12605),#3845,.F.);
#97579=ADVANCED_FACE('',(#12606),#6253,.F.);
#97580=ADVANCED_FACE('',(#12607),#92171,.F.);
#97581=ADVANCED_FACE('',(#12608),#3846,.F.);
#97582=ADVANCED_FACE('',(#12609),#92172,.F.);
#97583=ADVANCED_FACE('',(#12610),#92173,.F.);
#97584=ADVANCED_FACE('',(#12611),#3847,.F.);
#97585=ADVANCED_FACE('',(#12612),#3848,.F.);
#97586=ADVANCED_FACE('',(#12613),#92174,.F.);
#97587=ADVANCED_FACE('',(#12614),#92175,.F.);
#97588=ADVANCED_FACE('',(#12615),#3849,.F.);
#97589=ADVANCED_FACE('',(#12616),#92176,.F.);
#97590=ADVANCED_FACE('',(#12617),#92177,.F.);
#97591=ADVANCED_FACE('',(#12618),#3850,.F.);
#97592=ADVANCED_FACE('',(#12619),#92178,.F.);
#97593=ADVANCED_FACE('',(#12620),#92179,.F.);
#97594=ADVANCED_FACE('',(#12621),#3851,.F.);
#97595=ADVANCED_FACE('',(#12622),#3852,.F.);
#97596=ADVANCED_FACE('',(#12623),#92180,.F.);
#97597=ADVANCED_FACE('',(#12624),#92181,.F.);
#97598=ADVANCED_FACE('',(#12625),#3853,.F.);
#97599=ADVANCED_FACE('',(#12626),#92182,.F.);
#97600=ADVANCED_FACE('',(#12627),#6254,.F.);
#97601=ADVANCED_FACE('',(#12628),#3854,.F.);
#97602=ADVANCED_FACE('',(#12629),#3855,.F.);
#97603=ADVANCED_FACE('',(#12630),#92183,.F.);
#97604=ADVANCED_FACE('',(#12631),#92184,.F.);
#97605=ADVANCED_FACE('',(#12632),#3856,.F.);
#97606=ADVANCED_FACE('',(#12633),#3857,.F.);
#97607=ADVANCED_FACE('',(#12634),#6255,.F.);
#97608=ADVANCED_FACE('',(#12635),#92185,.F.);
#97609=ADVANCED_FACE('',(#12636),#3858,.F.);
#97610=ADVANCED_FACE('',(#12637),#92186,.F.);
#97611=ADVANCED_FACE('',(#12638),#92187,.F.);
#97612=ADVANCED_FACE('',(#12639),#3859,.F.);
#97613=ADVANCED_FACE('',(#12640),#3860,.F.);
#97614=ADVANCED_FACE('',(#12641),#92188,.F.);
#97615=ADVANCED_FACE('',(#12642),#92189,.F.);
#97616=ADVANCED_FACE('',(#12643),#3861,.F.);
#97617=ADVANCED_FACE('',(#12644),#92190,.F.);
#97618=ADVANCED_FACE('',(#12645),#92191,.F.);
#97619=ADVANCED_FACE('',(#12646),#3862,.F.);
#97620=ADVANCED_FACE('',(#12647),#92192,.F.);
#97621=ADVANCED_FACE('',(#12648),#92193,.F.);
#97622=ADVANCED_FACE('',(#12649),#3863,.F.);
#97623=ADVANCED_FACE('',(#12650),#3864,.F.);
#97624=ADVANCED_FACE('',(#12651),#92194,.F.);
#97625=ADVANCED_FACE('',(#12652),#92195,.F.);
#97626=ADVANCED_FACE('',(#12653),#3865,.F.);
#97627=ADVANCED_FACE('',(#12654),#92196,.F.);
#97628=ADVANCED_FACE('',(#12655),#6256,.F.);
#97629=ADVANCED_FACE('',(#12656),#3866,.F.);
#97630=ADVANCED_FACE('',(#12657),#3867,.F.);
#97631=ADVANCED_FACE('',(#12658),#92197,.F.);
#97632=ADVANCED_FACE('',(#12659),#92198,.F.);
#97633=ADVANCED_FACE('',(#12660),#3868,.F.);
#97634=ADVANCED_FACE('',(#12661),#3869,.F.);
#97635=ADVANCED_FACE('',(#12662),#6257,.F.);
#97636=ADVANCED_FACE('',(#12663),#92199,.F.);
#97637=ADVANCED_FACE('',(#12664),#3870,.F.);
#97638=ADVANCED_FACE('',(#12665),#92200,.F.);
#97639=ADVANCED_FACE('',(#12666),#92201,.F.);
#97640=ADVANCED_FACE('',(#12667),#3871,.F.);
#97641=ADVANCED_FACE('',(#12668),#3872,.F.);
#97642=ADVANCED_FACE('',(#12669),#92202,.F.);
#97643=ADVANCED_FACE('',(#12670),#92203,.F.);
#97644=ADVANCED_FACE('',(#12671),#3873,.F.);
#97645=ADVANCED_FACE('',(#12672),#92204,.F.);
#97646=ADVANCED_FACE('',(#12673),#92205,.F.);
#97647=ADVANCED_FACE('',(#12674),#3874,.F.);
#97648=ADVANCED_FACE('',(#12675),#92206,.F.);
#97649=ADVANCED_FACE('',(#12676),#92207,.F.);
#97650=ADVANCED_FACE('',(#12677),#3875,.F.);
#97651=ADVANCED_FACE('',(#12678),#3876,.F.);
#97652=ADVANCED_FACE('',(#12679),#92208,.F.);
#97653=ADVANCED_FACE('',(#12680),#92209,.F.);
#97654=ADVANCED_FACE('',(#12681),#3877,.F.);
#97655=ADVANCED_FACE('',(#12682),#92210,.F.);
#97656=ADVANCED_FACE('',(#12683),#6258,.F.);
#97657=ADVANCED_FACE('',(#12684),#3878,.F.);
#97658=ADVANCED_FACE('',(#12685),#3879,.F.);
#97659=ADVANCED_FACE('',(#12686),#92211,.F.);
#97660=ADVANCED_FACE('',(#12687),#92212,.F.);
#97661=ADVANCED_FACE('',(#12688),#3880,.F.);
#97662=ADVANCED_FACE('',(#12689),#3881,.F.);
#97663=ADVANCED_FACE('',(#12690),#6259,.F.);
#97664=ADVANCED_FACE('',(#12691),#92213,.F.);
#97665=ADVANCED_FACE('',(#12692),#3882,.F.);
#97666=ADVANCED_FACE('',(#12693),#92214,.F.);
#97667=ADVANCED_FACE('',(#12694),#92215,.F.);
#97668=ADVANCED_FACE('',(#12695),#3883,.F.);
#97669=ADVANCED_FACE('',(#12696),#3884,.F.);
#97670=ADVANCED_FACE('',(#12697),#92216,.F.);
#97671=ADVANCED_FACE('',(#12698),#92217,.F.);
#97672=ADVANCED_FACE('',(#12699),#3885,.F.);
#97673=ADVANCED_FACE('',(#12700),#92218,.F.);
#97674=ADVANCED_FACE('',(#12701),#92219,.F.);
#97675=ADVANCED_FACE('',(#12702),#3886,.F.);
#97676=ADVANCED_FACE('',(#12703),#92220,.F.);
#97677=ADVANCED_FACE('',(#12704),#92221,.F.);
#97678=ADVANCED_FACE('',(#12705),#3887,.F.);
#97679=ADVANCED_FACE('',(#12706),#3888,.F.);
#97680=ADVANCED_FACE('',(#12707),#92222,.F.);
#97681=ADVANCED_FACE('',(#12708),#92223,.F.);
#97682=ADVANCED_FACE('',(#12709),#3889,.F.);
#97683=ADVANCED_FACE('',(#12710),#92224,.F.);
#97684=ADVANCED_FACE('',(#12711),#6260,.F.);
#97685=ADVANCED_FACE('',(#12712),#3890,.F.);
#97686=ADVANCED_FACE('',(#12713),#3891,.F.);
#97687=ADVANCED_FACE('',(#12714),#92225,.F.);
#97688=ADVANCED_FACE('',(#12715),#92226,.F.);
#97689=ADVANCED_FACE('',(#12716),#3892,.F.);
#97690=ADVANCED_FACE('',(#12717),#3893,.F.);
#97691=ADVANCED_FACE('',(#12718),#6261,.F.);
#97692=ADVANCED_FACE('',(#12719),#92227,.F.);
#97693=ADVANCED_FACE('',(#12720),#3894,.F.);
#97694=ADVANCED_FACE('',(#12721),#92228,.F.);
#97695=ADVANCED_FACE('',(#12722),#92229,.F.);
#97696=ADVANCED_FACE('',(#12723),#3895,.F.);
#97697=ADVANCED_FACE('',(#12724),#3896,.F.);
#97698=ADVANCED_FACE('',(#12725),#92230,.F.);
#97699=ADVANCED_FACE('',(#12726),#92231,.F.);
#97700=ADVANCED_FACE('',(#12727),#3897,.F.);
#97701=ADVANCED_FACE('',(#12728),#92232,.F.);
#97702=ADVANCED_FACE('',(#12729),#92233,.F.);
#97703=ADVANCED_FACE('',(#12730),#3898,.F.);
#97704=ADVANCED_FACE('',(#12731),#92234,.F.);
#97705=ADVANCED_FACE('',(#12732),#92235,.F.);
#97706=ADVANCED_FACE('',(#12733),#3899,.F.);
#97707=ADVANCED_FACE('',(#12734),#3900,.F.);
#97708=ADVANCED_FACE('',(#12735),#92236,.F.);
#97709=ADVANCED_FACE('',(#12736),#92237,.F.);
#97710=ADVANCED_FACE('',(#12737),#3901,.F.);
#97711=ADVANCED_FACE('',(#12738),#92238,.F.);
#97712=ADVANCED_FACE('',(#12739),#6262,.F.);
#97713=ADVANCED_FACE('',(#12740),#3902,.F.);
#97714=ADVANCED_FACE('',(#12741),#3903,.F.);
#97715=ADVANCED_FACE('',(#12742),#92239,.F.);
#97716=ADVANCED_FACE('',(#12743),#92240,.F.);
#97717=ADVANCED_FACE('',(#12744),#3904,.F.);
#97718=ADVANCED_FACE('',(#12745),#3905,.F.);
#97719=ADVANCED_FACE('',(#12746),#6263,.F.);
#97720=ADVANCED_FACE('',(#12747),#92241,.F.);
#97721=ADVANCED_FACE('',(#12748),#3906,.F.);
#97722=ADVANCED_FACE('',(#12749),#92242,.F.);
#97723=ADVANCED_FACE('',(#12750),#92243,.F.);
#97724=ADVANCED_FACE('',(#12751),#3907,.F.);
#97725=ADVANCED_FACE('',(#12752),#3908,.F.);
#97726=ADVANCED_FACE('',(#12753),#92244,.F.);
#97727=ADVANCED_FACE('',(#12754),#92245,.F.);
#97728=ADVANCED_FACE('',(#12755),#3909,.F.);
#97729=ADVANCED_FACE('',(#12756),#92246,.F.);
#97730=ADVANCED_FACE('',(#12757),#92247,.F.);
#97731=ADVANCED_FACE('',(#12758),#3910,.F.);
#97732=ADVANCED_FACE('',(#12759),#92248,.F.);
#97733=ADVANCED_FACE('',(#12760),#92249,.F.);
#97734=ADVANCED_FACE('',(#12761),#3911,.F.);
#97735=ADVANCED_FACE('',(#12762),#3912,.F.);
#97736=ADVANCED_FACE('',(#12763),#92250,.F.);
#97737=ADVANCED_FACE('',(#12764),#92251,.F.);
#97738=ADVANCED_FACE('',(#12765),#3913,.F.);
#97739=ADVANCED_FACE('',(#12766),#92252,.F.);
#97740=ADVANCED_FACE('',(#12767),#6264,.F.);
#97741=ADVANCED_FACE('',(#12768),#3914,.F.);
#97742=ADVANCED_FACE('',(#12769),#3915,.F.);
#97743=ADVANCED_FACE('',(#12770),#92253,.F.);
#97744=ADVANCED_FACE('',(#12771),#92254,.F.);
#97745=ADVANCED_FACE('',(#12772),#3916,.F.);
#97746=ADVANCED_FACE('',(#12773),#3917,.F.);
#97747=ADVANCED_FACE('',(#12774),#6265,.F.);
#97748=ADVANCED_FACE('',(#12775),#92255,.F.);
#97749=ADVANCED_FACE('',(#12776),#3918,.F.);
#97750=ADVANCED_FACE('',(#12777),#92256,.F.);
#97751=ADVANCED_FACE('',(#12778),#92257,.F.);
#97752=ADVANCED_FACE('',(#12779),#3919,.F.);
#97753=ADVANCED_FACE('',(#12780),#3920,.F.);
#97754=ADVANCED_FACE('',(#12781),#92258,.F.);
#97755=ADVANCED_FACE('',(#12782),#92259,.F.);
#97756=ADVANCED_FACE('',(#12783),#3921,.F.);
#97757=ADVANCED_FACE('',(#12784),#92260,.F.);
#97758=ADVANCED_FACE('',(#12785),#92261,.F.);
#97759=ADVANCED_FACE('',(#12786),#3922,.F.);
#97760=ADVANCED_FACE('',(#12787),#92262,.F.);
#97761=ADVANCED_FACE('',(#12788),#92263,.F.);
#97762=ADVANCED_FACE('',(#12789),#3923,.F.);
#97763=ADVANCED_FACE('',(#12790),#3924,.F.);
#97764=ADVANCED_FACE('',(#12791),#92264,.F.);
#97765=ADVANCED_FACE('',(#12792),#92265,.F.);
#97766=ADVANCED_FACE('',(#12793),#3925,.F.);
#97767=ADVANCED_FACE('',(#12794),#92266,.F.);
#97768=ADVANCED_FACE('',(#12795),#6266,.F.);
#97769=ADVANCED_FACE('',(#12796),#3926,.F.);
#97770=ADVANCED_FACE('',(#12797),#3927,.F.);
#97771=ADVANCED_FACE('',(#12798),#92267,.F.);
#97772=ADVANCED_FACE('',(#12799),#92268,.F.);
#97773=ADVANCED_FACE('',(#12800),#3928,.F.);
#97774=ADVANCED_FACE('',(#12801),#3929,.F.);
#97775=ADVANCED_FACE('',(#12802),#6267,.F.);
#97776=ADVANCED_FACE('',(#12803),#92269,.F.);
#97777=ADVANCED_FACE('',(#12804),#3930,.F.);
#97778=ADVANCED_FACE('',(#12805),#92270,.F.);
#97779=ADVANCED_FACE('',(#12806),#92271,.F.);
#97780=ADVANCED_FACE('',(#12807),#3931,.F.);
#97781=ADVANCED_FACE('',(#12808),#3932,.F.);
#97782=ADVANCED_FACE('',(#12809),#92272,.F.);
#97783=ADVANCED_FACE('',(#12810),#92273,.F.);
#97784=ADVANCED_FACE('',(#12811),#3933,.F.);
#97785=ADVANCED_FACE('',(#12812),#92274,.F.);
#97786=ADVANCED_FACE('',(#12813),#92275,.F.);
#97787=ADVANCED_FACE('',(#12814),#3934,.F.);
#97788=ADVANCED_FACE('',(#12815),#92276,.F.);
#97789=ADVANCED_FACE('',(#12816),#92277,.F.);
#97790=ADVANCED_FACE('',(#12817),#3935,.F.);
#97791=ADVANCED_FACE('',(#12818),#3936,.F.);
#97792=ADVANCED_FACE('',(#12819),#92278,.F.);
#97793=ADVANCED_FACE('',(#12820),#92279,.F.);
#97794=ADVANCED_FACE('',(#12821),#3937,.F.);
#97795=ADVANCED_FACE('',(#12822),#92280,.F.);
#97796=ADVANCED_FACE('',(#12823),#6268,.F.);
#97797=ADVANCED_FACE('',(#12824),#3938,.F.);
#97798=ADVANCED_FACE('',(#12825),#3939,.F.);
#97799=ADVANCED_FACE('',(#12826),#92281,.F.);
#97800=ADVANCED_FACE('',(#12827),#92282,.F.);
#97801=ADVANCED_FACE('',(#12828),#3940,.F.);
#97802=ADVANCED_FACE('',(#12829),#3941,.F.);
#97803=ADVANCED_FACE('',(#12830),#6269,.F.);
#97804=ADVANCED_FACE('',(#12831),#92283,.F.);
#97805=ADVANCED_FACE('',(#12832),#3942,.F.);
#97806=ADVANCED_FACE('',(#12833),#92284,.F.);
#97807=ADVANCED_FACE('',(#12834),#92285,.F.);
#97808=ADVANCED_FACE('',(#12835),#3943,.F.);
#97809=ADVANCED_FACE('',(#12836),#3944,.F.);
#97810=ADVANCED_FACE('',(#12837),#92286,.F.);
#97811=ADVANCED_FACE('',(#12838),#92287,.F.);
#97812=ADVANCED_FACE('',(#12839),#3945,.F.);
#97813=ADVANCED_FACE('',(#12840),#92288,.F.);
#97814=ADVANCED_FACE('',(#12841),#6270,.T.);
#97815=ADVANCED_FACE('',(#12842),#6271,.F.);
#97816=ADVANCED_FACE('',(#12843),#6272,.T.);
#97817=ADVANCED_FACE('',(#12844),#92289,.F.);
#97818=ADVANCED_FACE('',(#12845),#92290,.F.);
#97819=ADVANCED_FACE('',(#12846),#92291,.T.);
#97820=ADVANCED_FACE('',(#12847,#6372),#7228,.T.);
#97821=ADVANCED_FACE('',(#12848,#6373),#7229,.F.);
#97822=ADVANCED_FACE('',(#12849,#6374),#7230,.T.);
#97823=ADVANCED_FACE('',(#12850),#6273,.T.);
#97824=ADVANCED_FACE('',(#12851),#6274,.T.);
#97825=ADVANCED_FACE('',(#12852),#92292,.F.);
#97826=ADVANCED_FACE('',(#12853),#92293,.T.);
#97827=ADVANCED_FACE('',(#12854,#6375),#7231,.F.);
#97828=ADVANCED_FACE('',(#12855,#6376),#7232,.T.);
#97829=ADVANCED_FACE('',(#12856),#6275,.T.);
#97830=ADVANCED_FACE('',(#12857),#6276,.T.);
#97831=ADVANCED_FACE('',(#12858),#6277,.T.);
#97832=ADVANCED_FACE('',(#12859),#6278,.T.);
#97833=ADVANCED_FACE('',(#12860),#3946,.T.);
#97834=ADVANCED_FACE('',(#12861),#3947,.T.);
#97835=ADVANCED_FACE('',(#12862),#3948,.T.);
#97836=ADVANCED_FACE('',(#12863),#6279,.F.);
#97837=ADVANCED_FACE('',(#12864),#3949,.T.);
#97838=ADVANCED_FACE('',(#12865),#92294,.F.);
#97839=ADVANCED_FACE('',(#12866),#92295,.F.);
#97840=ADVANCED_FACE('',(#12867),#6280,.T.);
#97841=ADVANCED_FACE('',(#12868),#92296,.F.);
#97842=ADVANCED_FACE('',(#12869),#92297,.F.);
#97843=ADVANCED_FACE('',(#12870),#92298,.F.);
#97844=ADVANCED_FACE('',(#12871),#92299,.F.);
#97845=ADVANCED_FACE('',(#12872),#92300,.F.);
#97846=ADVANCED_FACE('',(#12873),#92301,.T.);
#97847=ADVANCED_FACE('',(#12874),#312,.T.);
#97848=ADVANCED_FACE('',(#12875),#92302,.T.);
#97849=ADVANCED_FACE('',(#12876),#92303,.T.);
#97850=ADVANCED_FACE('',(#12877),#7233,.F.);
#97851=ADVANCED_FACE('',(#12878),#7234,.F.);
#97852=ADVANCED_FACE('',(#12879),#7235,.F.);
#97853=ADVANCED_FACE('',(#12880),#92304,.T.);
#97854=ADVANCED_FACE('',(#12881),#92305,.T.);
#97855=ADVANCED_FACE('',(#12882),#7236,.F.);
#97856=ADVANCED_FACE('',(#12883),#92306,.F.);
#97857=ADVANCED_FACE('',(#12884),#7237,.T.);
#97858=ADVANCED_FACE('',(#12885),#92307,.F.);
#97859=ADVANCED_FACE('',(#12886),#7238,.T.);
#97860=ADVANCED_FACE('',(#12887),#92308,.F.);
#97861=ADVANCED_FACE('',(#12888),#7239,.T.);
#97862=ADVANCED_FACE('',(#12889),#92309,.F.);
#97863=ADVANCED_FACE('',(#12890),#7240,.T.);
#97864=ADVANCED_FACE('',(#12891,#6377),#7241,.T.);
#97865=ADVANCED_FACE('',(#12892),#7242,.F.);
#97866=ADVANCED_FACE('',(#12893),#7243,.T.);
#97867=ADVANCED_FACE('',(#12894),#92310,.T.);
#97868=ADVANCED_FACE('',(#12895),#3950,.F.);
#97869=ADVANCED_FACE('',(#12896),#92311,.T.);
#97870=ADVANCED_FACE('',(#12897),#7244,.T.);
#97871=ADVANCED_FACE('',(#12898),#7245,.T.);
#97872=ADVANCED_FACE('',(#12899),#92312,.T.);
#97873=ADVANCED_FACE('',(#12900,#6378),#7246,.T.);
#97874=ADVANCED_FACE('',(#12901),#92313,.T.);
#97875=ADVANCED_FACE('',(#12902,#6379),#7247,.T.);
#97876=ADVANCED_FACE('',(#12903),#92314,.T.);
#97877=ADVANCED_FACE('',(#12904,#6380),#7248,.T.);
#97878=ADVANCED_FACE('',(#12905,#6381),#7249,.T.);
#97879=ADVANCED_FACE('',(#12906),#7250,.T.);
#97880=ADVANCED_FACE('',(#12907),#7251,.T.);
#97881=ADVANCED_FACE('',(#12908),#7252,.T.);
#97882=ADVANCED_FACE('',(#12909),#7253,.T.);
#97883=ADVANCED_FACE('',(#12910),#7254,.T.);
#97884=ADVANCED_FACE('',(#12911),#7255,.T.);
#97885=ADVANCED_FACE('',(#12912),#7256,.T.);
#97886=ADVANCED_FACE('',(#12913),#7257,.T.);
#97887=ADVANCED_FACE('',(#12914),#7258,.T.);
#97888=ADVANCED_FACE('',(#12915),#7259,.T.);
#97889=ADVANCED_FACE('',(#12916),#7260,.T.);
#97890=ADVANCED_FACE('',(#12917,#6382,#6383,#6384,#6385,#6386),#7261,.T.);
#97891=ADVANCED_FACE('',(#12918,#6387),#7262,.F.);
#97892=ADVANCED_FACE('',(#12919,#6388),#7263,.T.);
#97893=ADVANCED_FACE('',(#12920),#6281,.T.);
#97894=ADVANCED_FACE('',(#12921),#6282,.T.);
#97895=ADVANCED_FACE('',(#12922),#6283,.T.);
#97896=ADVANCED_FACE('',(#12923),#6284,.T.);
#97897=ADVANCED_FACE('',(#12924),#92315,.F.);
#97898=ADVANCED_FACE('',(#12925),#3951,.F.);
#97899=ADVANCED_FACE('',(#12926),#92316,.F.);
#97900=ADVANCED_FACE('',(#12927),#3952,.F.);
#97901=ADVANCED_FACE('',(#12928),#92317,.F.);
#97902=ADVANCED_FACE('',(#12929),#3953,.F.);
#97903=ADVANCED_FACE('',(#12930),#92318,.F.);
#97904=ADVANCED_FACE('',(#12931),#3954,.F.);
#97905=ADVANCED_FACE('',(#12932),#92319,.F.);
#97906=ADVANCED_FACE('',(#12933),#3955,.F.);
#97907=ADVANCED_FACE('',(#12934),#92320,.F.);
#97908=ADVANCED_FACE('',(#12935),#3956,.F.);
#97909=ADVANCED_FACE('',(#12936),#3957,.F.);
#97910=ADVANCED_FACE('',(#12937),#3958,.F.);
#97911=ADVANCED_FACE('',(#12938),#3959,.T.);
#97912=ADVANCED_FACE('',(#12939),#92321,.F.);
#97913=ADVANCED_FACE('',(#12940),#6285,.F.);
#97914=ADVANCED_FACE('',(#12941),#6286,.F.);
#97915=ADVANCED_FACE('',(#12942),#3960,.T.);
#97916=ADVANCED_FACE('',(#12943),#3961,.F.);
#97917=ADVANCED_FACE('',(#12944),#92322,.F.);
#97918=ADVANCED_FACE('',(#12945),#92323,.T.);
#97919=ADVANCED_FACE('',(#12946),#6287,.F.);
#97920=ADVANCED_FACE('',(#12947),#3962,.F.);
#97921=ADVANCED_FACE('',(#12948),#92324,.F.);
#97922=ADVANCED_FACE('',(#12949),#6288,.F.);
#97923=ADVANCED_FACE('',(#12950),#3963,.F.);
#97924=ADVANCED_FACE('',(#12951),#92325,.F.);
#97925=ADVANCED_FACE('',(#12952),#92326,.T.);
#97926=ADVANCED_FACE('',(#12953),#6289,.F.);
#97927=ADVANCED_FACE('',(#12954),#3964,.F.);
#97928=ADVANCED_FACE('',(#12955),#92327,.F.);
#97929=ADVANCED_FACE('',(#12956),#6290,.F.);
#97930=ADVANCED_FACE('',(#12957),#6291,.F.);
#97931=ADVANCED_FACE('',(#12958),#3965,.F.);
#97932=ADVANCED_FACE('',(#12959),#92328,.F.);
#97933=ADVANCED_FACE('',(#12960),#92329,.T.);
#97934=ADVANCED_FACE('',(#12961),#6292,.F.);
#97935=ADVANCED_FACE('',(#12962),#3966,.F.);
#97936=ADVANCED_FACE('',(#12963),#92330,.T.);
#97937=ADVANCED_FACE('',(#12964),#3967,.T.);
#97938=ADVANCED_FACE('',(#12965),#92331,.T.);
#97939=ADVANCED_FACE('',(#12966),#92332,.T.);
#97940=ADVANCED_FACE('',(#12967),#6293,.T.);
#97941=ADVANCED_FACE('',(#12968),#92333,.T.);
#97942=ADVANCED_FACE('',(#12969),#92334,.T.);
#97943=ADVANCED_FACE('',(#12970),#92335,.T.);
#97944=ADVANCED_FACE('',(#12971),#92336,.T.);
#97945=ADVANCED_FACE('',(#12972),#92337,.T.);
#97946=ADVANCED_FACE('',(#12973),#92338,.T.);
#97947=ADVANCED_FACE('',(#12974),#6294,.T.);
#97948=ADVANCED_FACE('',(#12975),#92339,.T.);
#97949=ADVANCED_FACE('',(#12976),#3968,.F.);
#97950=ADVANCED_FACE('',(#12977),#6295,.F.);
#97951=ADVANCED_FACE('',(#12978),#3969,.F.);
#97952=ADVANCED_FACE('',(#12979),#3970,.F.);
#97953=ADVANCED_FACE('',(#12980),#6296,.F.);
#97954=ADVANCED_FACE('',(#12981),#3971,.F.);
#97955=ADVANCED_FACE('',(#12982),#3972,.F.);
#97956=ADVANCED_FACE('',(#12983),#6297,.F.);
#97957=ADVANCED_FACE('',(#12984),#3973,.F.);
#97958=ADVANCED_FACE('',(#12985),#3974,.F.);
#97959=ADVANCED_FACE('',(#12986),#6298,.F.);
#97960=ADVANCED_FACE('',(#12987),#3975,.F.);
#97961=ADVANCED_FACE('',(#12988),#3976,.F.);
#97962=ADVANCED_FACE('',(#12989),#3977,.F.);
#97963=ADVANCED_FACE('',(#12990),#92340,.F.);
#97964=ADVANCED_FACE('',(#12991),#3978,.F.);
#97965=ADVANCED_FACE('',(#12992),#3979,.F.);
#97966=ADVANCED_FACE('',(#12993),#92341,.F.);
#97967=ADVANCED_FACE('',(#12994),#3980,.T.);
#97968=ADVANCED_FACE('',(#12995),#46,.T.);
#97969=ADVANCED_FACE('',(#12996),#3981,.T.);
#97970=ADVANCED_FACE('',(#12997),#47,.T.);
#97971=ADVANCED_FACE('',(#12998),#3982,.F.);
#97972=ADVANCED_FACE('',(#12999),#3983,.F.);
#97973=ADVANCED_FACE('',(#13000),#3984,.T.);
#97974=ADVANCED_FACE('',(#13001),#3985,.T.);
#97975=ADVANCED_FACE('',(#13002),#3986,.T.);
#97976=ADVANCED_FACE('',(#13003),#3987,.T.);
#97977=ADVANCED_FACE('',(#13004),#3988,.T.);
#97978=ADVANCED_FACE('',(#13005),#3989,.T.);
#97979=ADVANCED_FACE('',(#13006),#3990,.T.);
#97980=ADVANCED_FACE('',(#13007),#3991,.T.);
#97981=ADVANCED_FACE('',(#13008),#3992,.T.);
#97982=ADVANCED_FACE('',(#13009),#3993,.T.);
#97983=ADVANCED_FACE('',(#13010),#3994,.T.);
#97984=ADVANCED_FACE('',(#13011),#3995,.T.);
#97985=ADVANCED_FACE('',(#13012),#3996,.T.);
#97986=ADVANCED_FACE('',(#13013),#3997,.T.);
#97987=ADVANCED_FACE('',(#13014),#3998,.T.);
#97988=ADVANCED_FACE('',(#13015),#3999,.T.);
#97989=ADVANCED_FACE('',(#13016),#4000,.T.);
#97990=ADVANCED_FACE('',(#13017),#4001,.T.);
#97991=ADVANCED_FACE('',(#13018),#4002,.T.);
#97992=ADVANCED_FACE('',(#13019),#4003,.T.);
#97993=ADVANCED_FACE('',(#13020),#4004,.T.);
#97994=ADVANCED_FACE('',(#13021),#4005,.T.);
#97995=ADVANCED_FACE('',(#13022),#4006,.T.);
#97996=ADVANCED_FACE('',(#13023),#4007,.T.);
#97997=ADVANCED_FACE('',(#13024),#4008,.T.);
#97998=ADVANCED_FACE('',(#13025),#4009,.T.);
#97999=ADVANCED_FACE('',(#13026),#92342,.T.);
#98000=ADVANCED_FACE('',(#13027),#4010,.T.);
#98001=ADVANCED_FACE('',(#13028),#6299,.T.);
#98002=ADVANCED_FACE('',(#13029),#92343,.T.);
#98003=ADVANCED_FACE('',(#13030),#48,.T.);
#98004=ADVANCED_FACE('',(#13031),#6300,.T.);
#98005=ADVANCED_FACE('',(#13032),#6301,.T.);
#98006=ADVANCED_FACE('',(#13033),#4011,.T.);
#98007=ADVANCED_FACE('',(#13034),#92344,.F.);
#98008=ADVANCED_FACE('',(#13035),#92345,.T.);
#98009=ADVANCED_FACE('',(#13036),#92346,.T.);
#98010=ADVANCED_FACE('',(#13037),#49,.T.);
#98011=ADVANCED_FACE('',(#13038,#6389),#7264,.F.);
#98012=ADVANCED_FACE('',(#13039),#4012,.T.);
#98013=ADVANCED_FACE('',(#13040),#6302,.T.);
#98014=ADVANCED_FACE('',(#13041),#6303,.T.);
#98015=ADVANCED_FACE('',(#13042),#92347,.F.);
#98016=ADVANCED_FACE('',(#13043,#6390),#92348,.F.);
#98017=ADVANCED_FACE('',(#13044,#6391),#92349,.T.);
#98018=ADVANCED_FACE('',(#13045,#6392),#7265,.F.);
#98019=ADVANCED_FACE('',(#13046,#6393),#7266,.T.);
#98020=ADVANCED_FACE('',(#13047),#6304,.F.);
#98021=ADVANCED_FACE('',(#13048),#6305,.T.);
#98022=ADVANCED_FACE('',(#13049),#6306,.T.);
#98023=ADVANCED_FACE('',(#13050),#6307,.T.);
#98024=ADVANCED_FACE('',(#13051),#6308,.T.);
#98025=ADVANCED_FACE('',(#13052),#92350,.T.);
#98026=ADVANCED_FACE('',(#13053),#313,.F.);
#98027=ADVANCED_FACE('',(#13054),#314,.T.);
#98028=ADVANCED_FACE('',(#13055),#92351,.T.);
#98029=ADVANCED_FACE('',(#13056),#92352,.F.);
#98030=ADVANCED_FACE('',(#13057),#92353,.T.);
#98031=ADVANCED_FACE('',(#13058,#6394),#7267,.T.);
#98032=ADVANCED_FACE('',(#13059,#6395),#7268,.T.);
#98033=ADVANCED_FACE('',(#13060,#6396),#7269,.T.);
#98034=ADVANCED_FACE('',(#13061,#6397),#7270,.T.);
#98035=ADVANCED_FACE('',(#13062,#6398),#7271,.T.);
#98036=ADVANCED_FACE('',(#13063),#92354,.T.);
#98037=ADVANCED_FACE('',(#13064),#92355,.T.);
#98038=ADVANCED_FACE('',(#13065),#92356,.T.);
#98039=ADVANCED_FACE('',(#13066),#92357,.T.);
#98040=ADVANCED_FACE('',(#13067),#92358,.T.);
#98041=ADVANCED_FACE('',(#13068),#92359,.T.);
#98042=ADVANCED_FACE('',(#13069),#92360,.T.);
#98043=ADVANCED_FACE('',(#13070),#92361,.T.);
#98044=ADVANCED_FACE('',(#13071),#92362,.T.);
#98045=ADVANCED_FACE('',(#13072),#92363,.T.);
#98046=ADVANCED_FACE('',(#13073),#92364,.T.);
#98047=ADVANCED_FACE('',(#13074),#92365,.T.);
#98048=ADVANCED_FACE('',(#13075),#92366,.T.);
#98049=ADVANCED_FACE('',(#13076),#92367,.T.);
#98050=ADVANCED_FACE('',(#13077),#315,.T.);
#98051=ADVANCED_FACE('',(#13078),#316,.T.);
#98052=ADVANCED_FACE('',(#13079),#92368,.T.);
#98053=ADVANCED_FACE('',(#13080),#7272,.F.);
#98054=ADVANCED_FACE('',(#13081,#6399),#7273,.T.);
#98055=ADVANCED_FACE('',(#13082),#317,.F.);
#98056=ADVANCED_FACE('',(#13083),#318,.F.);
#98057=ADVANCED_FACE('',(#13084),#319,.F.);
#98058=ADVANCED_FACE('',(#13085),#320,.F.);
#98059=ADVANCED_FACE('',(#13086),#321,.F.);
#98060=ADVANCED_FACE('',(#13087),#322,.F.);
#98061=ADVANCED_FACE('',(#13088),#7274,.F.);
#98062=ADVANCED_FACE('',(#13089),#7275,.F.);
#98063=ADVANCED_FACE('',(#13090),#7276,.F.);
#98064=ADVANCED_FACE('',(#13091),#7277,.F.);
#98065=ADVANCED_FACE('',(#13092),#7278,.F.);
#98066=ADVANCED_FACE('',(#13093),#7279,.F.);
#98067=ADVANCED_FACE('',(#13094),#7280,.F.);
#98068=ADVANCED_FACE('',(#13095),#4013,.F.);
#98069=ADVANCED_FACE('',(#13096),#92369,.T.);
#98070=ADVANCED_FACE('',(#13097),#4014,.F.);
#98071=ADVANCED_FACE('',(#13098),#92370,.T.);
#98072=ADVANCED_FACE('',(#13099),#92371,.T.);
#98073=ADVANCED_FACE('',(#13100),#92372,.T.);
#98074=ADVANCED_FACE('',(#13101),#92373,.T.);
#98075=ADVANCED_FACE('',(#13102),#92374,.T.);
#98076=ADVANCED_FACE('',(#13103),#92375,.T.);
#98077=ADVANCED_FACE('',(#13104),#92376,.T.);
#98078=ADVANCED_FACE('',(#13105),#92377,.T.);
#98079=ADVANCED_FACE('',(#13106),#92378,.T.);
#98080=ADVANCED_FACE('',(#13107),#92379,.T.);
#98081=ADVANCED_FACE('',(#13108),#92380,.T.);
#98082=ADVANCED_FACE('',(#13109),#92381,.T.);
#98083=ADVANCED_FACE('',(#13110),#92382,.T.);
#98084=ADVANCED_FACE('',(#13111),#92383,.T.);
#98085=ADVANCED_FACE('',(#13112),#323,.T.);
#98086=ADVANCED_FACE('',(#13113),#324,.T.);
#98087=ADVANCED_FACE('',(#13114),#92384,.T.);
#98088=ADVANCED_FACE('',(#13115),#7281,.F.);
#98089=ADVANCED_FACE('',(#13116,#6400),#7282,.T.);
#98090=ADVANCED_FACE('',(#13117),#325,.F.);
#98091=ADVANCED_FACE('',(#13118),#326,.F.);
#98092=ADVANCED_FACE('',(#13119),#327,.F.);
#98093=ADVANCED_FACE('',(#13120),#328,.F.);
#98094=ADVANCED_FACE('',(#13121),#329,.F.);
#98095=ADVANCED_FACE('',(#13122),#330,.F.);
#98096=ADVANCED_FACE('',(#13123),#7283,.F.);
#98097=ADVANCED_FACE('',(#13124),#7284,.F.);
#98098=ADVANCED_FACE('',(#13125),#7285,.F.);
#98099=ADVANCED_FACE('',(#13126),#7286,.F.);
#98100=ADVANCED_FACE('',(#13127),#7287,.F.);
#98101=ADVANCED_FACE('',(#13128),#7288,.F.);
#98102=ADVANCED_FACE('',(#13129),#7289,.F.);
#98103=ADVANCED_FACE('',(#13130),#4015,.F.);
#98104=ADVANCED_FACE('',(#13131),#92385,.T.);
#98105=ADVANCED_FACE('',(#13132),#4016,.F.);
#98106=ADVANCED_FACE('',(#13133),#331,.F.);
#98107=ADVANCED_FACE('',(#13134),#332,.F.);
#98108=ADVANCED_FACE('',(#13135),#333,.T.);
#98109=ADVANCED_FACE('',(#13136),#334,.T.);
#98110=ADVANCED_FACE('',(#13137,#6401),#92386,.T.);
#98111=ADVANCED_FACE('',(#13138),#92387,.F.);
#98112=ADVANCED_FACE('',(#13139),#92388,.F.);
#98113=ADVANCED_FACE('',(#13140,#6402),#92389,.F.);
#98114=ADVANCED_FACE('',(#13141,#6403),#7290,.T.);
#98115=ADVANCED_FACE('',(#13142,#6404),#7291,.T.);
#98116=ADVANCED_FACE('',(#13143),#92390,.T.);
#98117=ADVANCED_FACE('',(#13144),#92391,.F.);
#98118=ADVANCED_FACE('',(#13145),#6309,.F.);
#98119=ADVANCED_FACE('',(#13146),#92392,.F.);
#98120=ADVANCED_FACE('',(#13147),#92393,.F.);
#98121=ADVANCED_FACE('',(#13148),#92394,.T.);
#98122=ADVANCED_FACE('',(#13149),#92395,.F.);
#98123=ADVANCED_FACE('',(#13150),#92396,.F.);
#98124=ADVANCED_FACE('',(#13151),#92397,.F.);
#98125=ADVANCED_FACE('',(#13152),#92398,.F.);
#98126=ADVANCED_FACE('',(#13153),#92399,.F.);
#98127=ADVANCED_FACE('',(#13154),#92400,.F.);
#98128=ADVANCED_FACE('',(#13155),#92401,.F.);
#98129=ADVANCED_FACE('',(#13156),#92402,.F.);
#98130=ADVANCED_FACE('',(#13157),#92403,.F.);
#98131=ADVANCED_FACE('',(#13158),#92404,.T.);
#98132=ADVANCED_FACE('',(#13159),#7292,.F.);
#98133=ADVANCED_FACE('',(#13160),#92405,.T.);
#98134=ADVANCED_FACE('',(#13161),#7293,.F.);
#98135=ADVANCED_FACE('',(#13162),#92406,.T.);
#98136=ADVANCED_FACE('',(#13163),#7294,.F.);
#98137=ADVANCED_FACE('',(#13164),#92407,.T.);
#98138=ADVANCED_FACE('',(#13165),#7295,.F.);
#98139=ADVANCED_FACE('',(#13166,#6405,#6406,#6407,#6408,#6409),#7296,.F.);
#98140=ADVANCED_FACE('',(#13167,#6410),#7297,.F.);
#98141=ADVANCED_FACE('',(#13168,#6411),#7298,.F.);
#98142=ADVANCED_FACE('',(#13169,#6412),#7299,.F.);
#98143=ADVANCED_FACE('',(#13170,#6413),#7300,.F.);
#98144=ADVANCED_FACE('',(#13171,#6414),#7301,.F.);
#98145=ADVANCED_FACE('',(#13172),#92408,.T.);
#98146=ADVANCED_FACE('',(#13173),#7302,.F.);
#98147=ADVANCED_FACE('',(#13174),#92409,.T.);
#98148=ADVANCED_FACE('',(#13175),#7303,.F.);
#98149=ADVANCED_FACE('',(#13176),#92410,.T.);
#98150=ADVANCED_FACE('',(#13177),#7304,.F.);
#98151=ADVANCED_FACE('',(#13178),#92411,.T.);
#98152=ADVANCED_FACE('',(#13179),#7305,.F.);
#98153=ADVANCED_FACE('',(#13180),#6310,.T.);
#98154=ADVANCED_FACE('',(#13181),#92412,.T.);
#98155=ADVANCED_FACE('',(#13182),#92413,.T.);
#98156=ADVANCED_FACE('',(#13183),#6311,.T.);
#98157=ADVANCED_FACE('',(#13184),#6312,.T.);
#98158=ADVANCED_FACE('',(#13185),#92414,.T.);
#98159=ADVANCED_FACE('',(#13186),#92415,.T.);
#98160=ADVANCED_FACE('',(#13187),#6313,.T.);
#98161=ADVANCED_FACE('',(#13188,#6415,#6416,#6417,#6418,#6419),#7306,.T.);
#98162=ADVANCED_FACE('',(#13189),#92416,.F.);
#98163=ADVANCED_FACE('',(#13190,#6420),#7307,.T.);
#98164=ADVANCED_FACE('',(#13191,#6421),#7308,.F.);
#98165=ADVANCED_FACE('',(#13192,#6422),#7309,.T.);
#98166=ADVANCED_FACE('',(#13193,#6423),#7310,.T.);
#98167=ADVANCED_FACE('',(#13194),#92417,.F.);
#98168=ADVANCED_FACE('',(#13195),#7311,.F.);
#98169=ADVANCED_FACE('',(#13196),#7312,.F.);
#98170=ADVANCED_FACE('',(#13197,#6424),#7313,.F.);
#98171=ADVANCED_FACE('',(#13198),#92418,.F.);
#98172=ADVANCED_FACE('',(#13199),#7314,.F.);
#98173=ADVANCED_FACE('',(#13200),#7315,.F.);
#98700=CLOSED_SHELL('',(#92680,#92681,#92682,#92683,#92684,#92685,#92686,
#92687,#92688,#92689,#92690,#92691,#92692,#92693,#92694,#92695,#92696,#92697,
#92698,#92699,#92700,#92701,#92702,#92703,#92704,#92705,#92706,#92707,#92708,
#92709,#92710,#92711,#92712,#92713,#92714,#92715));
#98701=CLOSED_SHELL('',(#92716,#92717,#92718,#92719));
#98702=CLOSED_SHELL('',(#92720,#92721,#92722,#92723));
#98703=CLOSED_SHELL('',(#92724,#92725,#92726,#92727));
#98704=CLOSED_SHELL('',(#92728,#92729,#92730,#92731));
#98705=CLOSED_SHELL('',(#92732,#92733,#92734,#92735,#92736,#92737));
#98706=CLOSED_SHELL('',(#92738,#92739,#92740,#92741,#92742,#92743));
#98707=CLOSED_SHELL('',(#92744,#92745,#92746,#92747));
#98708=CLOSED_SHELL('',(#92748,#92749,#92750,#92751,#92752,#92753,#92754,
#92755,#92756,#92757,#92758,#92759,#92760,#92761,#92762,#92763,#92764,#92765,
#92766,#92767,#92768,#92769,#92770,#92771,#92772,#92773,#92774,#92775,#92776,
#92777,#92778,#92779,#92780,#92781,#92782,#92783,#92784,#92785,#92786,#92787,
#92788,#92789,#92790,#92791,#92792,#92793,#92794,#92795,#92796,#92797,#92798,
#92799,#92800,#92801,#92802,#92803,#92804,#92805,#92806,#92807,#92808,#92809,
#92810,#92811,#92812,#92813,#92814,#92815,#92816,#92817,#92818,#92819,#92820,
#92821,#92822,#92823,#92824,#92825,#92826,#92827,#92828,#92829,#92830,#92831,
#92832,#92833,#92834,#92835,#92836,#92837,#92838,#92839,#92840,#92841,#92842,
#92843,#92844,#92845,#92846,#92847,#92848,#92849,#92850,#92851,#92852,#92853,
#92854,#92855,#92856,#92857,#92858,#92859,#92860,#92861,#92862,#92863,#92864,
#92865,#92866,#92867,#92868,#92869,#92870,#92871,#92872,#92873,#92874,#92875,
#92876,#92877,#92878,#92879,#92880,#92881,#92882,#92883,#92884,#92885,#92886,
#92887,#92888,#92889,#92890,#92891,#92892,#92893,#92894,#92895,#92896,#92897,
#92898,#92899,#92900,#92901,#92902,#92903,#92904,#92905,#92906,#92907,#92908,
#92909,#92910,#92911,#92912,#92913,#92914,#92915,#92916,#92917,#92918,#92919,
#92920,#92921,#92922,#92923,#92924,#92925,#92926,#92927,#92928,#92929,#92930,
#92931,#92932,#92933,#92934,#92935,#92936,#92937,#92938,#92939,#92940,#92941,
#92942,#92943,#92944,#92945,#92946,#92947,#92948,#92949,#92950,#92951,#92952,
#92953,#92954,#92955,#92956,#92957,#92958,#92959,#92960,#92961,#92962,#92963,
#92964,#92965,#92966,#92967,#92968,#92969,#92970,#92971,#92972,#92973,#92974,
#92975,#92976,#92977,#92978,#92979,#92980,#92981,#92982,#92983,#92984,#92985,
#92986,#92987,#92988,#92989,#92990,#92991,#92992,#92993,#92994,#92995,#92996,
#92997,#92998,#92999,#93000,#93001,#93002,#93003,#93004,#93005,#93006,#93007,
#93008,#93009,#93010,#93011,#93012,#93013,#93014,#93015,#93016,#93017,#93018,
#93019,#93020,#93021,#93022,#93023,#93024,#93025,#93026,#93027,#93028,#93029,
#93030,#93031,#93032,#93033,#93034,#93035,#93036,#93037,#93038,#93039,#93040,
#93041,#93042,#93043,#93044,#93045,#93046,#93047,#93048,#93049,#93050,#93051,
#93052,#93053,#93054,#93055,#93056,#93057,#93058,#93059,#93060,#93061,#93062,
#93063,#93064,#93065,#93066,#93067,#93068,#93069,#93070,#93071,#93072,#93073,
#93074,#93075,#93076,#93077,#93078,#93079,#93080,#93081,#93082,#93083,#93084,
#93085,#93086,#93087,#93088,#93089,#93090,#93091,#93092,#93093,#93094,#93095,
#93096,#93097,#93098,#93099,#93100,#93101,#93102,#93103,#93104,#93105,#93106,
#93107,#93108,#93109,#93110,#93111,#93112,#93113,#93114,#93115,#93116,#93117,
#93118,#93119,#93120,#93121,#93122,#93123,#93124,#93125,#93126,#93127,#93128,
#93129,#93130,#93131,#93132,#93133,#93134,#93135,#93136,#93137,#93138,#93139,
#93140,#93141,#93142,#93143,#93144,#93145,#93146,#93147,#93148,#93149,#93150,
#93151,#93152,#93153,#93154,#93155,#93156,#93157,#93158,#93159,#93160,#93161,
#93162,#93163,#93164,#93165,#93166,#93167,#93168,#93169,#93170,#93171,#93172,
#93173,#93174,#93175,#93176,#93177,#93178,#93179,#93180,#93181,#93182,#93183,
#93184,#93185,#93186,#93187,#93188,#93189,#93190,#93191,#93192,#93193,#93194,
#93195,#93196,#93197,#93198,#93199,#93200,#93201,#93202,#93203,#93204,#93205,
#93206,#93207,#93208,#93209,#93210,#93211,#93212,#93213,#93214,#93215,#93216,
#93217,#93218,#93219,#93220,#93221,#93222,#93223,#93224,#93225,#93226,#93227,
#93228,#93229,#93230,#93231,#93232,#93233,#93234,#93235,#93236,#93237,#93238,
#93239,#93240,#93241,#93242,#93243,#93244,#93245,#93246,#93247,#93248,#93249,
#93250,#93251,#93252,#93253,#93254,#93255,#93256,#93257,#93258,#93259,#93260,
#93261,#93262,#93263,#93264,#93265,#93266,#93267,#93268,#93269,#93270,#93271,
#93272,#93273,#93274,#93275,#93276,#93277,#93278,#93279,#93280,#93281,#93282,
#93283,#93284,#93285,#93286,#93287,#93288,#93289,#93290,#93291,#93292,#93293,
#93294,#93295,#93296,#93297,#93298,#93299,#93300,#93301,#93302,#93303,#93304,
#93305,#93306,#93307,#93308,#93309,#93310,#93311,#93312,#93313,#93314,#93315,
#93316,#93317,#93318,#93319,#93320,#93321,#93322,#93323,#93324,#93325,#93326,
#93327,#93328,#93329,#93330,#93331,#93332,#93333,#93334,#93335,#93336,#93337,
#93338,#93339,#93340,#93341,#93342,#93343,#93344,#93345,#93346,#93347,#93348,
#93349,#93350,#93351,#93352,#93353,#93354,#93355,#93356,#93357,#93358,#93359,
#93360,#93361,#93362,#93363,#93364,#93365,#93366,#93367,#93368,#93369,#93370,
#93371,#93372,#93373,#93374,#93375,#93376,#93377,#93378,#93379,#93380,#93381,
#93382,#93383,#93384,#93385,#93386,#93387,#93388,#93389,#93390,#93391,#93392,
#93393,#93394,#93395,#93396,#93397,#93398,#93399,#93400,#93401,#93402,#93403,
#93404,#93405,#93406,#93407,#93408,#93409,#93410,#93411,#93412,#93413,#93414,
#93415,#93416,#93417,#93418,#93419,#93420,#93421,#93422,#93423,#93424,#93425,
#93426,#93427,#93428,#93429,#93430,#93431,#93432,#93433,#93434,#93435,#93436,
#93437,#93438,#93439,#93440,#93441,#93442,#93443,#93444,#93445,#93446,#93447,
#93448,#93449,#93450,#93451,#93452,#93453,#93454,#93455,#93456,#93457,#93458,
#93459,#93460,#93461,#93462,#93463,#93464,#93465,#93466,#93467,#93468,#93469,
#93470,#93471,#93472,#93473,#93474,#93475,#93476,#93477,#93478,#93479,#93480,
#93481,#93482,#93483,#93484,#93485,#93486,#93487,#93488,#93489,#93490,#93491,
#93492,#93493,#93494,#93495,#93496,#93497,#93498,#93499,#93500,#93501,#93502,
#93503,#93504,#93505,#93506,#93507,#93508,#93509,#93510,#93511,#93512,#93513,
#93514,#93515,#93516,#93517,#93518,#93519,#93520,#93521,#93522,#93523,#93524,
#93525,#93526,#93527,#93528,#93529,#93530,#93531,#93532,#93533,#93534,#93535,
#93536,#93537,#93538,#93539,#93540,#93541,#93542,#93543,#93544,#93545,#93546,
#93547,#93548,#93549,#93550,#93551,#93552,#93553,#93554,#93555,#93556,#93557,
#93558,#93559,#93560,#93561,#93562,#93563,#93564,#93565,#93566,#93567,#93568,
#93569,#93570,#93571,#93572,#93573,#93574,#93575,#93576,#93577,#93578,#93579,
#93580,#93581,#93582,#93583,#93584,#93585,#93586,#93587,#93588,#93589,#93590,
#93591,#93592,#93593,#93594,#93595,#93596,#93597,#93598,#93599,#93600,#93601,
#93602,#93603,#93604,#93605,#93606,#93607,#93608,#93609,#93610,#93611,#93612,
#93613,#93614,#93615,#93616,#93617,#93618,#93619,#93620,#93621,#93622,#93623,
#93624,#93625,#93626,#93627,#93628,#93629,#93630,#93631,#93632,#93633,#93634,
#93635,#93636,#93637,#93638,#93639,#93640,#93641,#93642,#93643,#93644,#93645,
#93646,#93647,#93648,#93649,#93650,#93651,#93652,#93653,#93654,#93655,#93656,
#93657,#93658,#93659,#93660,#93661,#93662,#93663,#93664,#93665,#93666,#93667,
#93668,#93669,#93670,#93671,#93672,#93673,#93674,#93675,#93676,#93677,#93678,
#93679,#93680,#93681,#93682,#93683,#93684,#93685,#93686,#93687,#93688,#93689,
#93690,#93691,#93692,#93693,#93694,#93695,#93696,#93697,#93698,#93699,#93700,
#93701,#93702,#93703,#93704,#93705,#93706,#93707,#93708,#93709,#93710,#93711,
#93712,#93713,#93714,#93715,#93716,#93717,#93718,#93719,#93720,#93721,#93722,
#93723,#93724,#93725,#93726,#93727,#93728,#93729,#93730,#93731,#93732,#93733,
#93734,#93735,#93736,#93737,#93738,#93739,#93740,#93741,#93742,#93743,#93744,
#93745,#93746,#93747,#93748,#93749,#93750,#93751,#93752,#93753,#93754,#93755,
#93756,#93757,#93758,#93759,#93760,#93761,#93762,#93763,#93764,#93765,#93766,
#93767,#93768,#93769,#93770,#93771,#93772,#93773,#93774,#93775,#93776,#93777,
#93778,#93779,#93780,#93781,#93782,#93783,#93784,#93785,#93786,#93787,#93788,
#93789,#93790,#93791,#93792,#93793,#93794,#93795,#93796,#93797,#93798,#93799,
#93800,#93801,#93802,#93803,#93804,#93805,#93806,#93807,#93808,#93809,#93810,
#93811,#93812,#93813,#93814,#93815,#93816,#93817,#93818,#93819,#93820,#93821,
#93822,#93823,#93824,#93825,#93826,#93827,#93828,#93829,#93830,#93831,#93832,
#93833,#93834,#93835,#93836,#93837,#93838,#93839,#93840,#93841,#93842,#93843,
#93844,#93845,#93846,#93847,#93848,#93849,#93850,#93851,#93852,#93853,#93854,
#93855,#93856,#93857,#93858,#93859,#93860,#93861,#93862,#93863,#93864,#93865,
#93866,#93867,#93868,#93869,#93870,#93871,#93872,#93873,#93874,#93875,#93876,
#93877,#93878,#93879,#93880,#93881,#93882,#93883,#93884,#93885,#93886,#93887,
#93888,#93889,#93890,#93891,#93892,#93893,#93894,#93895,#93896,#93897,#93898,
#93899,#93900,#93901,#93902,#93903,#93904,#93905,#93906,#93907,#93908,#93909,
#93910,#93911,#93912,#93913,#93914,#93915,#93916,#93917,#93918,#93919,#93920,
#93921,#93922,#93923,#93924,#93925,#93926,#93927,#93928,#93929,#93930,#93931,
#93932,#93933,#93934,#93935,#93936,#93937,#93938,#93939,#93940,#93941,#93942,
#93943,#93944,#93945,#93946,#93947,#93948,#93949,#93950,#93951,#93952,#93953,
#93954,#93955,#93956,#93957,#93958,#93959,#93960,#93961,#93962,#93963,#93964,
#93965,#93966,#93967,#93968,#93969,#93970,#93971,#93972,#93973,#93974,#93975,
#93976,#93977,#93978,#93979,#93980,#93981,#93982,#93983,#93984,#93985,#93986,
#93987,#93988,#93989,#93990,#93991,#93992,#93993,#93994,#93995,#93996,#93997,
#93998,#93999,#94000,#94001,#94002,#94003,#94004,#94005,#94006,#94007,#94008,
#94009,#94010,#94011,#94012,#94013,#94014,#94015,#94016,#94017,#94018,#94019,
#94020,#94021,#94022,#94023,#94024,#94025,#94026,#94027,#94028,#94029,#94030,
#94031,#94032,#94033,#94034,#94035,#94036,#94037,#94038,#94039,#94040,#94041,
#94042,#94043,#94044,#94045,#94046,#94047,#94048,#94049,#94050,#94051,#94052,
#94053,#94054,#94055,#94056,#94057,#94058,#94059,#94060,#94061,#94062,#94063,
#94064,#94065,#94066,#94067,#94068,#94069,#94070,#94071,#94072,#94073,#94074,
#94075,#94076,#94077,#94078,#94079,#94080,#94081,#94082,#94083,#94084,#94085,
#94086,#94087,#94088,#94089,#94090,#94091,#94092,#94093,#94094,#94095,#94096,
#94097,#94098,#94099,#94100,#94101,#94102,#94103,#94104,#94105,#94106,#94107,
#94108,#94109,#94110,#94111,#94112,#94113,#94114,#94115,#94116,#94117,#94118,
#94119,#94120,#94121,#94122,#94123,#94124,#94125,#94126,#94127,#94128,#94129,
#94130,#94131,#94132,#94133,#94134,#94135,#94136,#94137,#94138,#94139,#94140,
#94141,#94142,#94143,#94144,#94145,#94146,#94147,#94148,#94149,#94150,#94151,
#94152,#94153,#94154,#94155,#94156,#94157,#94158,#94159,#94160,#94161,#94162,
#94163,#94164,#94165,#94166,#94167,#94168,#94169,#94170,#94171,#94172,#94173,
#94174,#94175,#94176,#94177,#94178,#94179,#94180,#94181,#94182,#94183,#94184,
#94185,#94186,#94187,#94188,#94189,#94190,#94191,#94192,#94193,#94194,#94195,
#94196,#94197,#94198,#94199,#94200,#94201,#94202,#94203,#94204,#94205,#94206,
#94207,#94208,#94209,#94210,#94211,#94212,#94213,#94214,#94215,#94216,#94217,
#94218,#94219,#94220,#94221,#94222,#94223,#94224,#94225,#94226,#94227,#94228,
#94229,#94230,#94231,#94232,#94233,#94234,#94235,#94236,#94237,#94238,#94239,
#94240,#94241,#94242,#94243,#94244,#94245,#94246,#94247,#94248,#94249,#94250,
#94251,#94252,#94253,#94254,#94255,#94256,#94257,#94258,#94259,#94260,#94261,
#94262,#94263,#94264,#94265,#94266,#94267,#94268,#94269,#94270,#94271,#94272,
#94273,#94274,#94275,#94276,#94277,#94278,#94279,#94280,#94281,#94282,#94283,
#94284,#94285,#94286,#94287,#94288,#94289,#94290,#94291,#94292,#94293,#94294,
#94295,#94296,#94297,#94298,#94299,#94300,#94301,#94302,#94303,#94304,#94305,
#94306,#94307,#94308,#94309,#94310,#94311,#94312,#94313,#94314,#94315,#94316,
#94317,#94318,#94319,#94320,#94321,#94322,#94323,#94324,#94325,#94326,#94327,
#94328,#94329,#94330,#94331,#94332,#94333,#94334,#94335,#94336,#94337,#94338,
#94339,#94340,#94341,#94342,#94343,#94344,#94345,#94346,#94347,#94348,#94349,
#94350,#94351,#94352,#94353,#94354,#94355,#94356,#94357,#94358,#94359,#94360,
#94361,#94362,#94363,#94364,#94365,#94366,#94367,#94368,#94369,#94370,#94371,
#94372,#94373,#94374,#94375,#94376,#94377,#94378,#94379,#94380,#94381,#94382,
#94383,#94384,#94385,#94386,#94387,#94388,#94389,#94390,#94391,#94392,#94393,
#94394,#94395,#94396,#94397,#94398,#94399,#94400,#94401,#94402,#94403,#94404,
#94405,#94406,#94407,#94408,#94409,#94410,#94411,#94412,#94413,#94414,#94415,
#94416,#94417,#94418,#94419,#94420,#94421,#94422,#94423,#94424,#94425,#94426,
#94427,#94428,#94429,#94430,#94431,#94432,#94433,#94434,#94435,#94436,#94437,
#94438,#94439,#94440,#94441,#94442,#94443,#94444,#94445,#94446,#94447,#94448,
#94449,#94450,#94451,#94452,#94453,#94454,#94455,#94456,#94457,#94458,#94459,
#94460,#94461,#94462,#94463,#94464,#94465,#94466,#94467,#94468,#94469,#94470,
#94471,#94472,#94473,#94474,#94475,#94476,#94477,#94478,#94479,#94480,#94481,
#94482,#94483,#94484,#94485,#94486,#94487,#94488,#94489,#94490,#94491,#94492,
#94493,#94494,#94495,#94496,#94497,#94498,#94499,#94500,#94501,#94502,#94503,
#94504,#94505,#94506,#94507,#94508,#94509,#94510,#94511,#94512,#94513,#94514,
#94515,#94516,#94517,#94518,#94519,#94520,#94521,#94522,#94523,#94524,#94525,
#94526,#94527,#94528,#94529,#94530,#94531,#94532,#94533,#94534,#94535,#94536,
#94537,#94538,#94539,#94540,#94541,#94542,#94543,#94544,#94545,#94546,#94547,
#94548,#94549,#94550,#94551,#94552,#94553,#94554,#94555,#94556,#94557,#94558,
#94559,#94560,#94561,#94562,#94563,#94564,#94565,#94566,#94567,#94568,#94569,
#94570,#94571,#94572,#94573,#94574,#94575,#94576,#94577,#94578,#94579,#94580,
#94581,#94582,#94583,#94584,#94585,#94586,#94587,#94588,#94589,#94590,#94591,
#94592,#94593,#94594,#94595,#94596,#94597,#94598,#94599,#94600,#94601,#94602,
#94603,#94604,#94605,#94606,#94607,#94608,#94609,#94610,#94611,#94612,#94613,
#94614,#94615,#94616,#94617,#94618,#94619,#94620,#94621,#94622,#94623,#94624,
#94625,#94626,#94627,#94628,#94629,#94630,#94631,#94632,#94633,#94634,#94635,
#94636,#94637,#94638,#94639,#94640,#94641,#94642,#94643,#94644,#94645,#94646,
#94647,#94648,#94649,#94650,#94651,#94652,#94653,#94654,#94655,#94656,#94657,
#94658,#94659,#94660,#94661,#94662,#94663,#94664,#94665,#94666,#94667,#94668,
#94669,#94670,#94671,#94672,#94673,#94674,#94675,#94676,#94677,#94678,#94679,
#94680,#94681,#94682,#94683,#94684,#94685,#94686,#94687,#94688,#94689,#94690,
#94691,#94692,#94693,#94694,#94695,#94696,#94697,#94698,#94699,#94700,#94701,
#94702,#94703,#94704,#94705,#94706,#94707,#94708,#94709,#94710,#94711,#94712,
#94713,#94714,#94715,#94716,#94717,#94718,#94719,#94720,#94721,#94722,#94723,
#94724,#94725,#94726,#94727,#94728,#94729,#94730,#94731,#94732,#94733,#94734,
#94735,#94736,#94737,#94738,#94739,#94740,#94741,#94742,#94743,#94744,#94745,
#94746,#94747,#94748,#94749,#94750,#94751,#94752,#94753,#94754,#94755,#94756,
#94757,#94758,#94759,#94760,#94761,#94762,#94763,#94764,#94765,#94766,#94767,
#94768,#94769,#94770,#94771,#94772,#94773,#94774,#94775,#94776,#94777,#94778,
#94779,#94780,#94781,#94782,#94783,#94784,#94785,#94786,#94787,#94788,#94789,
#94790,#94791,#94792,#94793,#94794,#94795,#94796,#94797,#94798,#94799,#94800,
#94801,#94802,#94803,#94804,#94805,#94806,#94807,#94808,#94809,#94810,#94811,
#94812,#94813,#94814,#94815,#94816,#94817,#94818,#94819,#94820,#94821,#94822,
#94823,#94824,#94825,#94826,#94827,#94828,#94829,#94830,#94831,#94832,#94833,
#94834,#94835,#94836,#94837,#94838,#94839,#94840,#94841,#94842,#94843,#94844,
#94845,#94846,#94847,#94848,#94849,#94850,#94851,#94852,#94853,#94854,#94855,
#94856,#94857,#94858,#94859,#94860,#94861,#94862,#94863,#94864,#94865,#94866,
#94867,#94868,#94869,#94870,#94871,#94872,#94873,#94874,#94875,#94876,#94877,
#94878,#94879,#94880,#94881,#94882,#94883,#94884,#94885,#94886,#94887,#94888,
#94889,#94890,#94891,#94892,#94893,#94894,#94895,#94896,#94897,#94898,#94899,
#94900,#94901,#94902,#94903,#94904,#94905,#94906,#94907,#94908,#94909,#94910,
#94911,#94912,#94913,#94914,#94915,#94916,#94917,#94918,#94919,#94920,#94921,
#94922,#94923,#94924,#94925,#94926,#94927,#94928,#94929,#94930,#94931,#94932,
#94933,#94934,#94935,#94936,#94937,#94938,#94939,#94940,#94941,#94942,#94943,
#94944,#94945,#94946,#94947,#94948,#94949,#94950,#94951,#94952,#94953,#94954,
#94955,#94956,#94957,#94958,#94959,#94960,#94961,#94962,#94963,#94964,#94965,
#94966,#94967,#94968,#94969,#94970,#94971,#94972,#94973,#94974,#94975,#94976,
#94977,#94978,#94979,#94980,#94981,#94982,#94983,#94984,#94985,#94986,#94987,
#94988,#94989,#94990,#94991,#94992,#94993,#94994,#94995,#94996,#94997,#94998,
#94999,#95000,#95001,#95002,#95003,#95004,#95005,#95006,#95007,#95008,#95009,
#95010,#95011,#95012,#95013,#95014,#95015,#95016,#95017,#95018,#95019,#95020,
#95021,#95022,#95023,#95024,#95025,#95026,#95027,#95028,#95029,#95030,#95031,
#95032,#95033,#95034,#95035,#95036,#95037,#95038,#95039,#95040,#95041,#95042,
#95043,#95044,#95045,#95046,#95047,#95048,#95049,#95050,#95051,#95052,#95053,
#95054,#95055,#95056,#95057,#95058,#95059,#95060,#95061,#95062,#95063,#95064,
#95065,#95066,#95067,#95068,#95069,#95070,#95071,#95072,#95073,#95074,#95075,
#95076,#95077,#95078,#95079,#95080,#95081,#95082,#95083,#95084,#95085,#95086,
#95087,#95088,#95089,#95090,#95091,#95092,#95093,#95094,#95095,#95096,#95097,
#95098,#95099,#95100,#95101,#95102,#95103,#95104,#95105,#95106,#95107,#95108,
#95109,#95110,#95111,#95112,#95113,#95114,#95115,#95116,#95117,#95118,#95119,
#95120,#95121,#95122,#95123,#95124,#95125,#95126,#95127,#95128,#95129,#95130,
#95131,#95132,#95133,#95134,#95135,#95136,#95137,#95138,#95139,#95140,#95141,
#95142,#95143,#95144,#95145,#95146,#95147,#95148,#95149,#95150,#95151,#95152,
#95153,#95154,#95155,#95156,#95157,#95158,#95159,#95160,#95161,#95162,#95163,
#95164,#95165,#95166,#95167,#95168,#95169,#95170,#95171,#95172,#95173,#95174,
#95175,#95176,#95177,#95178,#95179,#95180,#95181,#95182,#95183,#95184,#95185,
#95186,#95187,#95188,#95189,#95190,#95191,#95192,#95193,#95194,#95195,#95196,
#95197,#95198,#95199,#95200,#95201,#95202,#95203,#95204,#95205,#95206,#95207,
#95208,#95209,#95210,#95211,#95212,#95213,#95214,#95215,#95216,#95217,#95218,
#95219,#95220,#95221,#95222,#95223,#95224,#95225,#95226,#95227,#95228,#95229,
#95230,#95231,#95232,#95233,#95234,#95235,#95236,#95237,#95238,#95239,#95240,
#95241,#95242,#95243,#95244,#95245,#95246,#95247,#95248,#95249,#95250,#95251,
#95252,#95253,#95254,#95255,#95256,#95257,#95258,#95259,#95260,#95261,#95262,
#95263,#95264,#95265,#95266,#95267,#95268,#95269,#95270,#95271,#95272,#95273,
#95274,#95275,#95276,#95277,#95278,#95279,#95280));
#98709=CLOSED_SHELL('',(#95281,#95282,#95283,#95284,#95285,#95286,#95287,
#95288,#95289,#95290,#95291,#95292,#95293,#95294,#95295,#95296,#95297,#95298,
#95299,#95300,#95301,#95302,#95303,#95304,#95305,#95306,#95307,#95308,#95309,
#95310,#95311,#95312,#95313,#95314,#95315,#95316,#95317,#95318,#95319,#95320,
#95321,#95322,#95323,#95324,#95325,#95326,#95327,#95328,#95329,#95330,#95331,
#95332,#95333,#95334,#95335,#95336,#95337,#95338,#95339,#95340,#95341,#95342,
#95343,#95344,#95345,#95346,#95347,#95348,#95349,#95350,#95351,#95352,#95353,
#95354,#95355,#95356,#95357,#95358,#95359,#95360,#95361,#95362,#95363,#95364,
#95365,#95366,#95367,#95368,#95369,#95370,#95371,#95372,#95373,#95374,#95375,
#95376,#95377,#95378,#95379,#95380,#95381,#95382,#95383,#95384,#95385,#95386,
#95387,#95388,#95389,#95390,#95391,#95392,#95393,#95394,#95395,#95396,#95397,
#95398,#95399,#95400,#95401,#95402,#95403,#95404,#95405,#95406,#95407,#95408,
#95409,#95410,#95411,#95412,#95413,#95414,#95415,#95416,#95417,#95418,#95419,
#95420,#95421,#95422,#95423,#95424,#95425,#95426,#95427,#95428,#95429,#95430,
#95431,#95432,#95433,#95434,#95435,#95436,#95437,#95438,#95439,#95440,#95441,
#95442,#95443,#95444,#95445,#95446,#95447,#95448,#95449,#95450,#95451,#95452,
#95453,#95454,#95455,#95456,#95457,#95458,#95459,#95460,#95461,#95462,#95463,
#95464,#95465,#95466,#95467,#95468,#95469,#95470,#95471,#95472,#95473,#95474,
#95475,#95476,#95477,#95478,#95479,#95480,#95481,#95482,#95483,#95484,#95485,
#95486,#95487,#95488,#95489,#95490,#95491,#95492,#95493,#95494,#95495,#95496,
#95497,#95498,#95499,#95500,#95501,#95502,#95503,#95504,#95505,#95506,#95507,
#95508,#95509,#95510,#95511,#95512,#95513,#95514,#95515,#95516,#95517,#95518,
#95519,#95520,#95521,#95522,#95523,#95524,#95525,#95526,#95527,#95528,#95529,
#95530,#95531,#95532,#95533,#95534,#95535,#95536,#95537,#95538,#95539,#95540,
#95541,#95542,#95543,#95544,#95545,#95546,#95547,#95548,#95549,#95550,#95551,
#95552,#95553,#95554,#95555,#95556,#95557,#95558,#95559,#95560,#95561,#95562,
#95563,#95564,#95565,#95566,#95567,#95568,#95569,#95570,#95571,#95572,#95573,
#95574,#95575,#95576,#95577,#95578,#95579,#95580,#95581,#95582,#95583,#95584,
#95585,#95586,#95587,#95588,#95589,#95590,#95591,#95592,#95593,#95594,#95595,
#95596,#95597,#95598,#95599,#95600,#95601,#95602,#95603,#95604,#95605,#95606,
#95607,#95608,#95609,#95610,#95611,#95612,#95613,#95614,#95615,#95616,#95617,
#95618,#95619,#95620,#95621,#95622,#95623,#95624,#95625,#95626,#95627,#95628,
#95629,#95630,#95631,#95632,#95633,#95634,#95635,#95636,#95637,#95638,#95639,
#95640,#95641,#95642,#95643,#95644,#95645,#95646,#95647,#95648,#95649,#95650,
#95651,#95652,#95653,#95654,#95655,#95656,#95657,#95658,#95659,#95660,#95661,
#95662,#95663,#95664,#95665,#95666,#95667,#95668,#95669,#95670,#95671,#95672,
#95673,#95674,#95675,#95676,#95677,#95678,#95679,#95680,#95681,#95682,#95683,
#95684,#95685,#95686,#95687,#95688,#95689,#95690,#95691,#95692,#95693,#95694,
#95695,#95696,#95697,#95698,#95699,#95700,#95701,#95702,#95703,#95704,#95705,
#95706,#95707,#95708,#95709,#95710,#95711,#95712,#95713,#95714,#95715,#95716,
#95717,#95718,#95719,#95720,#95721,#95722,#95723,#95724,#95725,#95726,#95727,
#95728,#95729,#95730,#95731,#95732,#95733,#95734,#95735,#95736,#95737,#95738,
#95739,#95740,#95741,#95742,#95743,#95744,#95745,#95746,#95747,#95748,#95749,
#95750,#95751,#95752,#95753,#95754,#95755,#95756,#95757,#95758,#95759,#95760,
#95761,#95762,#95763,#95764,#95765,#95766,#95767,#95768,#95769,#95770,#95771,
#95772,#95773,#95774,#95775,#95776,#95777,#95778,#95779,#95780,#95781,#95782,
#95783,#95784,#95785,#95786,#95787,#95788,#95789,#95790,#95791,#95792,#95793,
#95794,#95795,#95796,#95797,#95798,#95799,#95800,#95801,#95802,#95803,#95804,
#95805,#95806,#95807,#95808,#95809,#95810,#95811,#95812,#95813,#95814,#95815,
#95816,#95817,#95818,#95819,#95820,#95821,#95822,#95823,#95824,#95825,#95826,
#95827,#95828,#95829,#95830,#95831,#95832,#95833,#95834,#95835,#95836,#95837,
#95838,#95839,#95840,#95841,#95842,#95843,#95844,#95845,#95846,#95847,#95848,
#95849,#95850,#95851,#95852,#95853,#95854,#95855,#95856,#95857,#95858,#95859,
#95860,#95861,#95862,#95863,#95864,#95865,#95866,#95867,#95868,#95869,#95870,
#95871,#95872,#95873,#95874,#95875,#95876,#95877,#95878,#95879,#95880,#95881,
#95882,#95883,#95884,#95885,#95886,#95887,#95888,#95889,#95890,#95891,#95892,
#95893,#95894,#95895,#95896,#95897,#95898,#95899,#95900,#95901,#95902,#95903,
#95904,#95905,#95906,#95907,#95908,#95909,#95910,#95911,#95912,#95913,#95914,
#95915,#95916,#95917,#95918,#95919,#95920,#95921,#95922,#95923,#95924,#95925,
#95926,#95927,#95928,#95929,#95930,#95931,#95932,#95933,#95934,#95935,#95936,
#95937,#95938,#95939,#95940,#95941,#95942,#95943,#95944,#95945,#95946,#95947,
#95948,#95949,#95950,#95951,#95952,#95953,#95954,#95955,#95956,#95957,#95958,
#95959,#95960,#95961,#95962,#95963,#95964,#95965,#95966,#95967,#95968,#95969,
#95970,#95971,#95972,#95973,#95974,#95975,#95976,#95977,#95978,#95979,#95980,
#95981,#95982,#95983,#95984,#95985,#95986,#95987,#95988,#95989,#95990,#95991,
#95992,#95993,#95994,#95995,#95996,#95997,#95998,#95999,#96000,#96001,#96002,
#96003,#96004,#96005,#96006,#96007,#96008,#96009,#96010,#96011,#96012,#96013,
#96014,#96015,#96016,#96017,#96018,#96019,#96020,#96021,#96022,#96023,#96024,
#96025,#96026,#96027,#96028,#96029,#96030,#96031,#96032,#96033,#96034,#96035,
#96036,#96037,#96038,#96039,#96040,#96041,#96042,#96043,#96044,#96045,#96046,
#96047,#96048,#96049,#96050,#96051,#96052,#96053,#96054,#96055,#96056,#96057,
#96058,#96059,#96060,#96061,#96062,#96063,#96064,#96065,#96066,#96067,#96068,
#96069,#96070,#96071,#96072,#96073,#96074,#96075,#96076,#96077,#96078,#96079,
#96080,#96081,#96082,#96083,#96084,#96085,#96086,#96087,#96088,#96089,#96090,
#96091,#96092,#96093,#96094,#96095,#96096,#96097,#96098,#96099,#96100,#96101,
#96102,#96103,#96104,#96105,#96106,#96107,#96108,#96109,#96110,#96111,#96112,
#96113,#96114,#96115,#96116,#96117,#96118,#96119,#96120,#96121,#96122,#96123,
#96124,#96125,#96126,#96127,#96128,#96129,#96130,#96131,#96132,#96133,#96134,
#96135,#96136,#96137,#96138,#96139,#96140,#96141,#96142,#96143,#96144,#96145,
#96146,#96147,#96148,#96149,#96150,#96151,#96152,#96153,#96154,#96155,#96156,
#96157,#96158,#96159,#96160,#96161,#96162,#96163,#96164,#96165,#96166,#96167,
#96168,#96169,#96170,#96171,#96172,#96173,#96174,#96175,#96176,#96177,#96178,
#96179,#96180,#96181,#96182,#96183,#96184,#96185,#96186,#96187,#96188,#96189,
#96190,#96191,#96192,#96193,#96194,#96195,#96196,#96197,#96198,#96199,#96200,
#96201,#96202,#96203,#96204,#96205,#96206,#96207,#96208,#96209,#96210,#96211,
#96212,#96213,#96214,#96215,#96216,#96217,#96218,#96219,#96220,#96221,#96222,
#96223,#96224,#96225,#96226,#96227,#96228,#96229,#96230,#96231,#96232,#96233,
#96234,#96235,#96236,#96237,#96238,#96239,#96240,#96241,#96242,#96243,#96244,
#96245,#96246,#96247,#96248,#96249,#96250,#96251,#96252,#96253,#96254,#96255,
#96256,#96257,#96258,#96259,#96260,#96261,#96262,#96263,#96264,#96265,#96266,
#96267,#96268,#96269,#96270,#96271,#96272,#96273,#96274,#96275,#96276,#96277,
#96278,#96279,#96280,#96281,#96282,#96283,#96284,#96285,#96286,#96287,#96288,
#96289,#96290,#96291,#96292,#96293,#96294,#96295,#96296,#96297,#96298,#96299,
#96300,#96301,#96302,#96303,#96304,#96305,#96306,#96307,#96308,#96309,#96310,
#96311,#96312,#96313,#96314,#96315,#96316,#96317,#96318,#96319,#96320,#96321,
#96322,#96323,#96324,#96325,#96326,#96327,#96328,#96329,#96330,#96331,#96332,
#96333,#96334,#96335,#96336,#96337,#96338,#96339,#96340,#96341,#96342,#96343,
#96344,#96345,#96346,#96347,#96348,#96349,#96350,#96351,#96352,#96353,#96354,
#96355,#96356,#96357,#96358,#96359,#96360,#96361,#96362,#96363,#96364,#96365,
#96366,#96367,#96368,#96369,#96370,#96371,#96372,#96373,#96374,#96375,#96376,
#96377,#96378,#96379,#96380,#96381,#96382,#96383,#96384,#96385,#96386,#96387,
#96388,#96389,#96390,#96391,#96392,#96393,#96394,#96395,#96396,#96397,#96398,
#96399,#96400,#96401,#96402,#96403,#96404,#96405,#96406,#96407,#96408,#96409,
#96410,#96411,#96412,#96413,#96414,#96415,#96416,#96417,#96418,#96419,#96420,
#96421,#96422,#96423,#96424,#96425,#96426,#96427,#96428,#96429,#96430,#96431,
#96432,#96433,#96434,#96435,#96436,#96437,#96438,#96439,#96440,#96441,#96442,
#96443,#96444,#96445,#96446,#96447,#96448,#96449,#96450,#96451,#96452,#96453,
#96454,#96455,#96456,#96457,#96458,#96459,#96460,#96461,#96462,#96463,#96464,
#96465,#96466,#96467,#96468,#96469,#96470,#96471,#96472,#96473,#96474,#96475,
#96476,#96477,#96478,#96479,#96480,#96481,#96482,#96483,#96484,#96485,#96486,
#96487,#96488,#96489,#96490,#96491,#96492,#96493,#96494,#96495,#96496,#96497,
#96498,#96499,#96500,#96501,#96502,#96503,#96504,#96505,#96506,#96507,#96508,
#96509,#96510,#96511,#96512,#96513,#96514,#96515,#96516,#96517,#96518,#96519,
#96520,#96521,#96522,#96523,#96524,#96525,#96526,#96527,#96528,#96529,#96530,
#96531,#96532,#96533,#96534,#96535,#96536,#96537,#96538,#96539,#96540,#96541,
#96542,#96543,#96544,#96545,#96546,#96547,#96548,#96549,#96550,#96551,#96552,
#96553,#96554,#96555,#96556,#96557,#96558,#96559,#96560,#96561,#96562,#96563,
#96564,#96565,#96566,#96567,#96568,#96569,#96570,#96571,#96572,#96573,#96574,
#96575,#96576,#96577,#96578,#96579,#96580,#96581,#96582,#96583,#96584,#96585,
#96586,#96587,#96588,#96589,#96590,#96591,#96592,#96593,#96594,#96595,#96596,
#96597,#96598,#96599,#96600,#96601,#96602,#96603,#96604,#96605,#96606,#96607,
#96608,#96609,#96610,#96611,#96612,#96613,#96614,#96615,#96616,#96617,#96618,
#96619,#96620,#96621,#96622,#96623,#96624,#96625,#96626,#96627,#96628,#96629,
#96630,#96631,#96632,#96633,#96634,#96635,#96636,#96637,#96638,#96639,#96640,
#96641,#96642,#96643,#96644,#96645,#96646,#96647,#96648,#96649,#96650,#96651,
#96652,#96653,#96654,#96655,#96656,#96657,#96658,#96659,#96660,#96661,#96662,
#96663,#96664,#96665,#96666,#96667,#96668,#96669,#96670,#96671,#96672,#96673,
#96674,#96675,#96676,#96677,#96678,#96679,#96680,#96681,#96682,#96683,#96684,
#96685,#96686,#96687,#96688,#96689,#96690,#96691,#96692,#96693,#96694,#96695,
#96696,#96697,#96698,#96699,#96700,#96701,#96702,#96703,#96704,#96705,#96706,
#96707,#96708,#96709,#96710,#96711,#96712,#96713,#96714,#96715,#96716,#96717,
#96718,#96719,#96720,#96721,#96722,#96723,#96724,#96725,#96726,#96727,#96728,
#96729,#96730,#96731,#96732,#96733,#96734,#96735,#96736,#96737,#96738,#96739,
#96740,#96741,#96742,#96743,#96744,#96745,#96746,#96747,#96748,#96749,#96750,
#96751,#96752,#96753,#96754,#96755,#96756,#96757,#96758,#96759,#96760,#96761,
#96762,#96763,#96764,#96765,#96766,#96767,#96768,#96769,#96770,#96771,#96772,
#96773,#96774,#96775,#96776,#96777,#96778,#96779,#96780,#96781,#96782,#96783,
#96784,#96785,#96786,#96787,#96788,#96789,#96790,#96791,#96792,#96793,#96794,
#96795,#96796,#96797,#96798,#96799,#96800,#96801,#96802,#96803,#96804,#96805,
#96806,#96807,#96808,#96809,#96810,#96811,#96812,#96813,#96814,#96815,#96816,
#96817,#96818,#96819,#96820,#96821,#96822,#96823,#96824,#96825,#96826,#96827,
#96828,#96829,#96830,#96831,#96832,#96833,#96834,#96835,#96836,#96837,#96838,
#96839,#96840,#96841,#96842,#96843,#96844,#96845,#96846,#96847,#96848,#96849,
#96850,#96851,#96852,#96853,#96854,#96855,#96856,#96857,#96858,#96859,#96860,
#96861,#96862,#96863,#96864,#96865,#96866,#96867,#96868,#96869,#96870,#96871,
#96872,#96873,#96874,#96875,#96876,#96877,#96878,#96879,#96880,#96881,#96882,
#96883,#96884,#96885,#96886,#96887,#96888,#96889,#96890,#96891,#96892,#96893,
#96894,#96895,#96896,#96897,#96898,#96899,#96900,#96901,#96902,#96903,#96904,
#96905,#96906,#96907,#96908,#96909,#96910,#96911,#96912,#96913,#96914,#96915,
#96916,#96917,#96918,#96919,#96920,#96921,#96922,#96923,#96924,#96925,#96926,
#96927,#96928,#96929,#96930,#96931,#96932,#96933,#96934,#96935,#96936,#96937,
#96938,#96939,#96940,#96941,#96942,#96943,#96944,#96945,#96946,#96947,#96948,
#96949,#96950,#96951,#96952,#96953,#96954,#96955,#96956,#96957,#96958,#96959,
#96960,#96961,#96962,#96963,#96964,#96965,#96966,#96967,#96968,#96969,#96970,
#96971,#96972,#96973,#96974,#96975,#96976,#96977,#96978,#96979,#96980,#96981,
#96982,#96983,#96984,#96985,#96986,#96987,#96988,#96989,#96990,#96991,#96992,
#96993,#96994,#96995,#96996,#96997,#96998,#96999,#97000,#97001,#97002,#97003,
#97004,#97005,#97006,#97007,#97008,#97009,#97010,#97011,#97012,#97013,#97014,
#97015,#97016,#97017,#97018,#97019,#97020,#97021,#97022,#97023,#97024,#97025,
#97026,#97027,#97028,#97029,#97030,#97031,#97032,#97033,#97034,#97035,#97036,
#97037,#97038,#97039,#97040,#97041,#97042,#97043,#97044,#97045,#97046,#97047,
#97048,#97049,#97050,#97051,#97052,#97053,#97054,#97055,#97056,#97057,#97058,
#97059,#97060,#97061,#97062,#97063,#97064,#97065,#97066,#97067,#97068,#97069,
#97070,#97071,#97072,#97073,#97074,#97075,#97076,#97077,#97078,#97079,#97080,
#97081,#97082,#97083,#97084,#97085,#97086,#97087,#97088,#97089,#97090,#97091,
#97092,#97093,#97094,#97095,#97096,#97097,#97098,#97099,#97100,#97101,#97102,
#97103,#97104,#97105,#97106,#97107,#97108,#97109,#97110,#97111,#97112,#97113,
#97114,#97115,#97116,#97117,#97118,#97119,#97120,#97121,#97122,#97123,#97124,
#97125,#97126,#97127,#97128,#97129,#97130,#97131,#97132,#97133,#97134,#97135,
#97136,#97137,#97138,#97139,#97140,#97141,#97142,#97143,#97144,#97145,#97146,
#97147,#97148,#97149,#97150,#97151,#97152,#97153,#97154,#97155,#97156,#97157,
#97158,#97159,#97160,#97161,#97162,#97163,#97164,#97165,#97166,#97167,#97168,
#97169,#97170,#97171,#97172,#97173,#97174,#97175,#97176,#97177,#97178,#97179,
#97180,#97181,#97182,#97183,#97184,#97185,#97186,#97187,#97188,#97189,#97190,
#97191,#97192,#97193,#97194,#97195,#97196,#97197,#97198,#97199,#97200,#97201,
#97202,#97203,#97204,#97205,#97206,#97207,#97208,#97209,#97210,#97211,#97212,
#97213,#97214,#97215,#97216,#97217,#97218,#97219,#97220,#97221,#97222,#97223,
#97224,#97225,#97226,#97227,#97228,#97229,#97230,#97231,#97232,#97233,#97234,
#97235,#97236,#97237,#97238,#97239,#97240,#97241,#97242,#97243,#97244,#97245,
#97246,#97247,#97248,#97249,#97250,#97251,#97252,#97253,#97254,#97255,#97256,
#97257,#97258,#97259,#97260,#97261,#97262,#97263,#97264,#97265,#97266,#97267,
#97268,#97269,#97270,#97271,#97272,#97273,#97274,#97275,#97276,#97277,#97278,
#97279,#97280,#97281,#97282,#97283,#97284,#97285,#97286,#97287,#97288,#97289,
#97290,#97291,#97292,#97293,#97294,#97295,#97296,#97297,#97298,#97299,#97300,
#97301,#97302,#97303,#97304,#97305,#97306,#97307,#97308,#97309,#97310,#97311,
#97312,#97313,#97314,#97315,#97316,#97317,#97318,#97319,#97320,#97321,#97322,
#97323,#97324,#97325,#97326,#97327,#97328,#97329,#97330,#97331,#97332,#97333,
#97334,#97335,#97336,#97337,#97338,#97339,#97340,#97341,#97342,#97343,#97344,
#97345,#97346,#97347,#97348,#97349,#97350,#97351,#97352,#97353,#97354,#97355,
#97356,#97357,#97358,#97359,#97360,#97361,#97362,#97363,#97364,#97365,#97366,
#97367,#97368,#97369,#97370,#97371,#97372,#97373,#97374,#97375,#97376,#97377,
#97378,#97379,#97380,#97381,#97382,#97383,#97384,#97385,#97386,#97387,#97388,
#97389,#97390,#97391,#97392,#97393,#97394,#97395,#97396,#97397,#97398,#97399,
#97400,#97401,#97402,#97403,#97404,#97405,#97406,#97407,#97408,#97409,#97410,
#97411,#97412,#97413,#97414,#97415,#97416,#97417,#97418,#97419,#97420,#97421,
#97422,#97423,#97424,#97425,#97426,#97427,#97428,#97429,#97430,#97431,#97432,
#97433,#97434,#97435,#97436,#97437,#97438,#97439,#97440,#97441,#97442,#97443,
#97444,#97445,#97446,#97447,#97448,#97449,#97450,#97451,#97452,#97453,#97454,
#97455,#97456,#97457,#97458,#97459,#97460,#97461,#97462,#97463,#97464,#97465,
#97466,#97467,#97468,#97469,#97470,#97471,#97472,#97473,#97474,#97475,#97476,
#97477,#97478,#97479,#97480,#97481,#97482,#97483,#97484,#97485,#97486,#97487,
#97488,#97489,#97490,#97491,#97492,#97493,#97494,#97495,#97496,#97497,#97498,
#97499,#97500,#97501,#97502,#97503,#97504,#97505,#97506,#97507,#97508,#97509,
#97510,#97511,#97512,#97513,#97514,#97515,#97516,#97517,#97518,#97519,#97520,
#97521,#97522,#97523,#97524,#97525,#97526,#97527,#97528,#97529,#97530,#97531,
#97532,#97533,#97534,#97535,#97536,#97537,#97538,#97539,#97540,#97541,#97542,
#97543,#97544,#97545,#97546,#97547,#97548,#97549,#97550,#97551,#97552,#97553,
#97554,#97555,#97556,#97557,#97558,#97559,#97560,#97561,#97562,#97563,#97564,
#97565,#97566,#97567,#97568,#97569,#97570,#97571,#97572,#97573,#97574,#97575,
#97576,#97577,#97578,#97579,#97580,#97581,#97582,#97583,#97584,#97585,#97586,
#97587,#97588,#97589,#97590,#97591,#97592,#97593,#97594,#97595,#97596,#97597,
#97598,#97599,#97600,#97601,#97602,#97603,#97604,#97605,#97606,#97607,#97608,
#97609,#97610,#97611,#97612,#97613,#97614,#97615,#97616,#97617,#97618,#97619,
#97620,#97621,#97622,#97623,#97624,#97625,#97626,#97627,#97628,#97629,#97630,
#97631,#97632,#97633,#97634,#97635,#97636,#97637,#97638,#97639,#97640,#97641,
#97642,#97643,#97644,#97645,#97646,#97647,#97648,#97649,#97650,#97651,#97652,
#97653,#97654,#97655,#97656,#97657,#97658,#97659,#97660,#97661,#97662,#97663,
#97664,#97665,#97666,#97667,#97668,#97669,#97670,#97671,#97672,#97673,#97674,
#97675,#97676,#97677,#97678,#97679,#97680,#97681,#97682,#97683,#97684,#97685,
#97686,#97687,#97688,#97689,#97690,#97691,#97692,#97693,#97694,#97695,#97696,
#97697,#97698,#97699,#97700,#97701,#97702,#97703,#97704,#97705,#97706,#97707,
#97708,#97709,#97710,#97711,#97712,#97713,#97714,#97715,#97716,#97717,#97718,
#97719,#97720,#97721,#97722,#97723,#97724,#97725,#97726,#97727,#97728,#97729,
#97730,#97731,#97732,#97733,#97734,#97735,#97736,#97737,#97738,#97739,#97740,
#97741,#97742,#97743,#97744,#97745,#97746,#97747,#97748,#97749,#97750,#97751,
#97752,#97753,#97754,#97755,#97756,#97757,#97758,#97759,#97760,#97761,#97762,
#97763,#97764,#97765,#97766,#97767,#97768,#97769,#97770,#97771,#97772,#97773,
#97774,#97775,#97776,#97777,#97778,#97779,#97780,#97781,#97782,#97783,#97784,
#97785,#97786,#97787,#97788,#97789,#97790,#97791,#97792,#97793,#97794,#97795,
#97796,#97797,#97798,#97799,#97800,#97801,#97802,#97803,#97804,#97805,#97806,
#97807,#97808,#97809,#97810,#97811,#97812,#97813));
#98710=CLOSED_SHELL('',(#97814,#97815,#97816,#97817,#97818,#97819,#97820,
#97821,#97822));
#98711=CLOSED_SHELL('',(#97823,#97824,#97825,#97826,#97827,#97828));
#98712=CLOSED_SHELL('',(#97829,#97830,#97831,#97832,#97833,#97834,#97835,
#97836,#97837,#97838,#97839,#97840,#97841,#97842,#97843,#97844,#97845,#97846,
#97847,#97848,#97849,#97850,#97851,#97852,#97853,#97854,#97855,#97856,#97857,
#97858,#97859,#97860,#97861,#97862,#97863,#97864,#97865,#97866,#97867,#97868,
#97869,#97870,#97871,#97872,#97873,#97874,#97875,#97876,#97877,#97878,#97879,
#97880,#97881,#97882,#97883,#97884,#97885,#97886,#97887,#97888,#97889,#97890,
#97891,#97892,#97893,#97894,#97895,#97896,#97897,#97898,#97899,#97900,#97901,
#97902,#97903,#97904,#97905,#97906,#97907,#97908,#97909,#97910,#97911,#97912,
#97913,#97914,#97915,#97916,#97917,#97918,#97919,#97920,#97921,#97922,#97923,
#97924,#97925,#97926,#97927,#97928,#97929,#97930,#97931,#97932,#97933,#97934,
#97935,#97936,#97937,#97938,#97939,#97940,#97941,#97942,#97943,#97944,#97945,
#97946,#97947,#97948,#97949,#97950,#97951,#97952,#97953,#97954,#97955,#97956,
#97957,#97958,#97959,#97960,#97961,#97962,#97963,#97964,#97965,#97966,#97967,
#97968,#97969,#97970,#97971,#97972,#97973,#97974,#97975,#97976,#97977,#97978,
#97979,#97980,#97981,#97982,#97983,#97984,#97985,#97986,#97987,#97988,#97989,
#97990,#97991,#97992,#97993,#97994,#97995,#97996,#97997,#97998,#97999,#98000,
#98001,#98002));
#98713=CLOSED_SHELL('',(#98003));
#98714=CLOSED_SHELL('',(#98004,#98005,#98006,#98007,#98008,#98009,#98010,
#98011,#98012));
#98715=CLOSED_SHELL('',(#98013,#98014,#98015,#98016,#98017,#98018,#98019));
#98716=CLOSED_SHELL('',(#98020,#98021,#98022,#98023,#98024,#98025,#98026,
#98027,#98028,#98029,#98030,#98031,#98032,#98033,#98034,#98035));
#98717=CLOSED_SHELL('',(#98036,#98037,#98038,#98039,#98040,#98041,#98042,
#98043,#98044,#98045,#98046,#98047,#98048,#98049,#98050,#98051,#98052,#98053,
#98054,#98055,#98056,#98057,#98058,#98059,#98060,#98061,#98062,#98063,#98064,
#98065,#98066,#98067,#98068,#98069,#98070));
#98718=CLOSED_SHELL('',(#98071,#98072,#98073,#98074,#98075,#98076,#98077,
#98078,#98079,#98080,#98081,#98082,#98083,#98084,#98085,#98086,#98087,#98088,
#98089,#98090,#98091,#98092,#98093,#98094,#98095,#98096,#98097,#98098,#98099,
#98100,#98101,#98102,#98103,#98104,#98105));
#98719=CLOSED_SHELL('',(#98106,#98107,#98108,#98109,#98110,#98111,#98112,
#98113,#98114,#98115));
#98720=CLOSED_SHELL('',(#98116,#98117,#98118,#98119,#98120,#98121,#98122,
#98123,#98124,#98125,#98126,#98127,#98128,#98129,#98130,#98131,#98132,#98133,
#98134,#98135,#98136,#98137,#98138,#98139,#98140,#98141,#98142,#98143,#98144,
#98145,#98146,#98147,#98148,#98149,#98150,#98151,#98152,#98153,#98154,#98155,
#98156,#98157,#98158,#98159,#98160,#98161,#98162,#98163,#98164,#98165,#98166,
#98167,#98168,#98169,#98170,#98171,#98172,#98173));
#98939=AXIS2_PLACEMENT_3D('',#167144,#112067,#112068);
#98940=AXIS2_PLACEMENT_3D('',#167145,#112069,#112070);
#98941=AXIS2_PLACEMENT_3D('',#167147,#112071,#112072);
#98942=AXIS2_PLACEMENT_3D('',#167149,#112073,#112074);
#98943=AXIS2_PLACEMENT_3D('',#167151,#112075,#112076);
#98944=AXIS2_PLACEMENT_3D('',#167152,#112077,#112078);
#98945=AXIS2_PLACEMENT_3D('',#167153,#112079,#112080);
#98946=AXIS2_PLACEMENT_3D('',#167180,#112083,#112084);
#98947=AXIS2_PLACEMENT_3D('',#167183,#112085,#112086);
#98948=AXIS2_PLACEMENT_3D('',#167190,#112087,#112088);
#98949=AXIS2_PLACEMENT_3D('',#167192,#112089,#112090);
#98950=AXIS2_PLACEMENT_3D('',#167195,#112092,#112093);
#98951=AXIS2_PLACEMENT_3D('',#167196,#112094,#112095);
#98952=AXIS2_PLACEMENT_3D('',#167199,#112096,#112097);
#98953=AXIS2_PLACEMENT_3D('',#167219,#112098,#112099);
#98954=AXIS2_PLACEMENT_3D('',#167220,#112100,#112101);
#98955=AXIS2_PLACEMENT_3D('',#167223,#112102,#112103);
#98956=AXIS2_PLACEMENT_3D('',#167225,#112104,#112105);
#98957=AXIS2_PLACEMENT_3D('',#167226,#112106,#112107);
#98958=AXIS2_PLACEMENT_3D('',#167229,#112109,#112110);
#98959=AXIS2_PLACEMENT_3D('',#167230,#112111,#112112);
#98960=AXIS2_PLACEMENT_3D('',#167231,#112113,#112114);
#98961=AXIS2_PLACEMENT_3D('',#167233,#112115,#112116);
#98962=AXIS2_PLACEMENT_3D('',#167234,#112117,#112118);
#98963=AXIS2_PLACEMENT_3D('',#167237,#112119,#112120);
#98964=AXIS2_PLACEMENT_3D('',#167238,#112121,#112122);
#98965=AXIS2_PLACEMENT_3D('',#167239,#112123,#112124);
#98966=AXIS2_PLACEMENT_3D('',#167240,#112125,#112126);
#98967=AXIS2_PLACEMENT_3D('',#167244,#112128,#112129);
#98968=AXIS2_PLACEMENT_3D('',#167245,#112130,#112131);
#98969=AXIS2_PLACEMENT_3D('',#167246,#112132,#112133);
#98970=AXIS2_PLACEMENT_3D('',#167248,#112134,#112135);
#98971=AXIS2_PLACEMENT_3D('',#167249,#112136,#112137);
#98972=AXIS2_PLACEMENT_3D('',#167250,#112138,#112139);
#98973=AXIS2_PLACEMENT_3D('',#167252,#112140,#112141);
#98974=AXIS2_PLACEMENT_3D('',#167255,#112143,#112144);
#98975=AXIS2_PLACEMENT_3D('',#167256,#112145,#112146);
#98976=AXIS2_PLACEMENT_3D('',#167257,#112147,#112148);
#98977=AXIS2_PLACEMENT_3D('',#167258,#112149,#112150);
#98978=AXIS2_PLACEMENT_3D('',#167265,#112151,#112152);
#98979=AXIS2_PLACEMENT_3D('',#167284,#112153,#112154);
#98980=AXIS2_PLACEMENT_3D('',#167303,#112155,#112156);
#98981=AXIS2_PLACEMENT_3D('',#167322,#112157,#112158);
#98982=AXIS2_PLACEMENT_3D('',#167341,#112159,#112160);
#98983=AXIS2_PLACEMENT_3D('',#167342,#112161,#112162);
#98984=AXIS2_PLACEMENT_3D('',#167344,#112163,#112164);
#98985=AXIS2_PLACEMENT_3D('',#167346,#112165,#112166);
#98986=AXIS2_PLACEMENT_3D('',#167348,#112167,#112168);
#98987=AXIS2_PLACEMENT_3D('',#167350,#112169,#112170);
#98988=AXIS2_PLACEMENT_3D('',#167351,#112171,#112172);
#98989=AXIS2_PLACEMENT_3D('',#167352,#112173,#112174);
#98990=AXIS2_PLACEMENT_3D('',#167371,#112175,#112176);
#98991=AXIS2_PLACEMENT_3D('',#167390,#112177,#112178);
#98992=AXIS2_PLACEMENT_3D('',#167409,#112179,#112180);
#98993=AXIS2_PLACEMENT_3D('',#167428,#112181,#112182);
#98994=AXIS2_PLACEMENT_3D('',#167447,#112183,#112184);
#98995=AXIS2_PLACEMENT_3D('',#167449,#112186,#112187);
#98996=AXIS2_PLACEMENT_3D('',#167452,#112190,#112191);
#98997=AXIS2_PLACEMENT_3D('',#167455,#112194,#112195);
#98998=AXIS2_PLACEMENT_3D('',#167458,#112198,#112199);
#98999=AXIS2_PLACEMENT_3D('',#167461,#112202,#112203);
#99000=AXIS2_PLACEMENT_3D('',#167463,#112205,#112206);
#99001=AXIS2_PLACEMENT_3D('',#167464,#112207,#112208);
#99002=AXIS2_PLACEMENT_3D('',#167465,#112209,#112210);
#99003=AXIS2_PLACEMENT_3D('',#167466,#112211,#112212);
#99004=AXIS2_PLACEMENT_3D('',#167467,#112213,#112214);
#99005=AXIS2_PLACEMENT_3D('',#167468,#112215,#112216);
#99006=AXIS2_PLACEMENT_3D('',#167470,#112217,#112218);
#99007=AXIS2_PLACEMENT_3D('',#167473,#112220,#112221);
#99008=AXIS2_PLACEMENT_3D('',#167474,#112222,#112223);
#99009=AXIS2_PLACEMENT_3D('',#167476,#112224,#112225);
#99010=AXIS2_PLACEMENT_3D('',#167479,#112227,#112228);
#99011=AXIS2_PLACEMENT_3D('',#167480,#112229,#112230);
#99012=AXIS2_PLACEMENT_3D('',#167481,#112231,#112232);
#99013=AXIS2_PLACEMENT_3D('',#167482,#112233,#112234);
#99014=AXIS2_PLACEMENT_3D('',#167484,#112235,#112236);
#99015=AXIS2_PLACEMENT_3D('',#167487,#112238,#112239);
#99016=AXIS2_PLACEMENT_3D('',#167488,#112240,#112241);
#99017=AXIS2_PLACEMENT_3D('',#167490,#112242,#112243);
#99018=AXIS2_PLACEMENT_3D('',#167493,#112245,#112246);
#99019=AXIS2_PLACEMENT_3D('',#167494,#112247,#112248);
#99020=AXIS2_PLACEMENT_3D('',#167495,#112249,#112250);
#99021=AXIS2_PLACEMENT_3D('',#167496,#112251,#112252);
#99022=AXIS2_PLACEMENT_3D('',#167498,#112253,#112254);
#99023=AXIS2_PLACEMENT_3D('',#167501,#112256,#112257);
#99024=AXIS2_PLACEMENT_3D('',#167502,#112258,#112259);
#99025=AXIS2_PLACEMENT_3D('',#167504,#112260,#112261);
#99026=AXIS2_PLACEMENT_3D('',#167507,#112263,#112264);
#99027=AXIS2_PLACEMENT_3D('',#167508,#112265,#112266);
#99028=AXIS2_PLACEMENT_3D('',#167509,#112267,#112268);
#99029=AXIS2_PLACEMENT_3D('',#167510,#112269,#112270);
#99030=AXIS2_PLACEMENT_3D('',#167512,#112271,#112272);
#99031=AXIS2_PLACEMENT_3D('',#167515,#112274,#112275);
#99032=AXIS2_PLACEMENT_3D('',#167516,#112276,#112277);
#99033=AXIS2_PLACEMENT_3D('',#167518,#112278,#112279);
#99034=AXIS2_PLACEMENT_3D('',#167521,#112281,#112282);
#99035=AXIS2_PLACEMENT_3D('',#167522,#112283,#112284);
#99036=AXIS2_PLACEMENT_3D('',#167523,#112285,#112286);
#99037=AXIS2_PLACEMENT_3D('',#167524,#112287,#112288);
#99038=AXIS2_PLACEMENT_3D('',#167527,#112289,#112290);
#99039=AXIS2_PLACEMENT_3D('',#167528,#112291,#112292);
#99040=AXIS2_PLACEMENT_3D('',#167530,#112293,#112294);
#99041=AXIS2_PLACEMENT_3D('',#167531,#112295,#112296);
#99042=AXIS2_PLACEMENT_3D('',#167532,#112297,#112298);
#99043=AXIS2_PLACEMENT_3D('',#167534,#112299,#112300);
#99044=AXIS2_PLACEMENT_3D('',#167536,#112301,#112302);
#99045=AXIS2_PLACEMENT_3D('',#167538,#112303,#112304);
#99046=AXIS2_PLACEMENT_3D('',#167539,#112305,#112306);
#99047=AXIS2_PLACEMENT_3D('',#167540,#112307,#112308);
#99048=AXIS2_PLACEMENT_3D('',#167542,#112309,#112310);
#99049=AXIS2_PLACEMENT_3D('',#167544,#112312,#112313);
#99050=AXIS2_PLACEMENT_3D('',#167547,#112315,#112316);
#99051=AXIS2_PLACEMENT_3D('',#167548,#112317,#112318);
#99052=AXIS2_PLACEMENT_3D('',#167549,#112319,#112320);
#99053=AXIS2_PLACEMENT_3D('',#167550,#112321,#112322);
#99054=AXIS2_PLACEMENT_3D('',#167552,#112323,#112324);
#99055=AXIS2_PLACEMENT_3D('',#167554,#112325,#112326);
#99056=AXIS2_PLACEMENT_3D('',#167556,#112327,#112328);
#99057=AXIS2_PLACEMENT_3D('',#167557,#112329,#112330);
#99058=AXIS2_PLACEMENT_3D('',#167558,#112331,#112332);
#99059=AXIS2_PLACEMENT_3D('',#167561,#112333,#112334);
#99060=AXIS2_PLACEMENT_3D('',#167562,#112335,#112336);
#99061=AXIS2_PLACEMENT_3D('',#167564,#112337,#112338);
#99062=AXIS2_PLACEMENT_3D('',#167565,#112339,#112340);
#99063=AXIS2_PLACEMENT_3D('',#167566,#112341,#112342);
#99064=AXIS2_PLACEMENT_3D('',#167568,#112343,#112344);
#99065=AXIS2_PLACEMENT_3D('',#167570,#112346,#112347);
#99066=AXIS2_PLACEMENT_3D('',#167573,#112349,#112350);
#99067=AXIS2_PLACEMENT_3D('',#167574,#112351,#112352);
#99068=AXIS2_PLACEMENT_3D('',#167575,#112353,#112354);
#99069=AXIS2_PLACEMENT_3D('',#167576,#112355,#112356);
#99070=AXIS2_PLACEMENT_3D('',#167578,#112357,#112358);
#99071=AXIS2_PLACEMENT_3D('',#167581,#112360,#112361);
#99072=AXIS2_PLACEMENT_3D('',#167582,#112362,#112363);
#99073=AXIS2_PLACEMENT_3D('',#167584,#112364,#112365);
#99074=AXIS2_PLACEMENT_3D('',#167587,#112367,#112368);
#99075=AXIS2_PLACEMENT_3D('',#167588,#112369,#112370);
#99076=AXIS2_PLACEMENT_3D('',#167589,#112371,#112372);
#99077=AXIS2_PLACEMENT_3D('',#167590,#112373,#112374);
#99078=AXIS2_PLACEMENT_3D('',#167593,#112375,#112376);
#99079=AXIS2_PLACEMENT_3D('',#167595,#112377,#112378);
#99080=AXIS2_PLACEMENT_3D('',#167597,#112379,#112380);
#99081=AXIS2_PLACEMENT_3D('',#167598,#112381,#112382);
#99082=AXIS2_PLACEMENT_3D('',#167599,#112383,#112384);
#99083=AXIS2_PLACEMENT_3D('',#167602,#112385,#112386);
#99084=AXIS2_PLACEMENT_3D('',#167604,#112387,#112388);
#99085=AXIS2_PLACEMENT_3D('',#167606,#112389,#112390);
#99086=AXIS2_PLACEMENT_3D('',#167607,#112391,#112392);
#99087=AXIS2_PLACEMENT_3D('',#167608,#112393,#112394);
#99088=AXIS2_PLACEMENT_3D('',#167611,#112395,#112396);
#99089=AXIS2_PLACEMENT_3D('',#167613,#112397,#112398);
#99090=AXIS2_PLACEMENT_3D('',#167615,#112399,#112400);
#99091=AXIS2_PLACEMENT_3D('',#167616,#112401,#112402);
#99092=AXIS2_PLACEMENT_3D('',#167617,#112403,#112404);
#99093=AXIS2_PLACEMENT_3D('',#167620,#112405,#112406);
#99094=AXIS2_PLACEMENT_3D('',#167622,#112407,#112408);
#99095=AXIS2_PLACEMENT_3D('',#167624,#112409,#112410);
#99096=AXIS2_PLACEMENT_3D('',#167626,#112411,#112412);
#99097=AXIS2_PLACEMENT_3D('',#167627,#112413,#112414);
#99098=AXIS2_PLACEMENT_3D('',#167628,#112415,#112416);
#99099=AXIS2_PLACEMENT_3D('',#167630,#112417,#112418);
#99100=AXIS2_PLACEMENT_3D('',#167632,#112419,#112420);
#99101=AXIS2_PLACEMENT_3D('',#167634,#112421,#112422);
#99102=AXIS2_PLACEMENT_3D('',#167635,#112423,#112424);
#99103=AXIS2_PLACEMENT_3D('',#167636,#112425,#112426);
#99104=AXIS2_PLACEMENT_3D('',#167638,#112427,#112428);
#99105=AXIS2_PLACEMENT_3D('',#167640,#112429,#112430);
#99106=AXIS2_PLACEMENT_3D('',#167641,#112431,#112432);
#99107=AXIS2_PLACEMENT_3D('',#167642,#112433,#112434);
#99108=AXIS2_PLACEMENT_3D('',#167644,#112435,#112436);
#99109=AXIS2_PLACEMENT_3D('',#167646,#112437,#112438);
#99110=AXIS2_PLACEMENT_3D('',#167648,#112439,#112440);
#99111=AXIS2_PLACEMENT_3D('',#167649,#112441,#112442);
#99112=AXIS2_PLACEMENT_3D('',#167650,#112443,#112444);
#99113=AXIS2_PLACEMENT_3D('',#167652,#112445,#112446);
#99114=AXIS2_PLACEMENT_3D('',#167654,#112447,#112448);
#99115=AXIS2_PLACEMENT_3D('',#167655,#112449,#112450);
#99116=AXIS2_PLACEMENT_3D('',#167656,#112451,#112452);
#99117=AXIS2_PLACEMENT_3D('',#167658,#112453,#112454);
#99118=AXIS2_PLACEMENT_3D('',#167661,#112456,#112457);
#99119=AXIS2_PLACEMENT_3D('',#167662,#112458,#112459);
#99120=AXIS2_PLACEMENT_3D('',#167664,#112461,#112462);
#99121=AXIS2_PLACEMENT_3D('',#167667,#112463,#112464);
#99122=AXIS2_PLACEMENT_3D('',#167715,#112466,#112467);
#99123=AXIS2_PLACEMENT_3D('',#167760,#112469,#112470);
#99124=AXIS2_PLACEMENT_3D('',#167808,#112472,#112473);
#99125=AXIS2_PLACEMENT_3D('',#167853,#112475,#112476);
#99126=AXIS2_PLACEMENT_3D('',#167901,#112478,#112479);
#99127=AXIS2_PLACEMENT_3D('',#167946,#112481,#112482);
#99128=AXIS2_PLACEMENT_3D('',#167994,#112484,#112485);
#99129=AXIS2_PLACEMENT_3D('',#168039,#112487,#112488);
#99130=AXIS2_PLACEMENT_3D('',#168087,#112490,#112491);
#99131=AXIS2_PLACEMENT_3D('',#168132,#112493,#112494);
#99132=AXIS2_PLACEMENT_3D('',#168180,#112496,#112497);
#99133=AXIS2_PLACEMENT_3D('',#168225,#112499,#112500);
#99134=AXIS2_PLACEMENT_3D('',#168273,#112502,#112503);
#99135=AXIS2_PLACEMENT_3D('',#168318,#112505,#112506);
#99136=AXIS2_PLACEMENT_3D('',#168366,#112508,#112509);
#99137=AXIS2_PLACEMENT_3D('',#168411,#112511,#112512);
#99138=AXIS2_PLACEMENT_3D('',#168459,#112514,#112515);
#99139=AXIS2_PLACEMENT_3D('',#168504,#112517,#112518);
#99140=AXIS2_PLACEMENT_3D('',#168552,#112520,#112521);
#99141=AXIS2_PLACEMENT_3D('',#168597,#112523,#112524);
#99142=AXIS2_PLACEMENT_3D('',#168645,#112526,#112527);
#99143=AXIS2_PLACEMENT_3D('',#168690,#112529,#112530);
#99144=AXIS2_PLACEMENT_3D('',#168738,#112532,#112533);
#99145=AXIS2_PLACEMENT_3D('',#168783,#112535,#112536);
#99146=AXIS2_PLACEMENT_3D('',#168831,#112538,#112539);
#99147=AXIS2_PLACEMENT_3D('',#168876,#112541,#112542);
#99148=AXIS2_PLACEMENT_3D('',#168924,#112544,#112545);
#99149=AXIS2_PLACEMENT_3D('',#168969,#112547,#112548);
#99150=AXIS2_PLACEMENT_3D('',#169017,#112550,#112551);
#99151=AXIS2_PLACEMENT_3D('',#169062,#112553,#112554);
#99152=AXIS2_PLACEMENT_3D('',#169110,#112556,#112557);
#99153=AXIS2_PLACEMENT_3D('',#169155,#112559,#112560);
#99154=AXIS2_PLACEMENT_3D('',#169203,#112562,#112563);
#99155=AXIS2_PLACEMENT_3D('',#169248,#112565,#112566);
#99156=AXIS2_PLACEMENT_3D('',#169296,#112568,#112569);
#99157=AXIS2_PLACEMENT_3D('',#169341,#112571,#112572);
#99158=AXIS2_PLACEMENT_3D('',#169389,#112574,#112575);
#99159=AXIS2_PLACEMENT_3D('',#169434,#112577,#112578);
#99160=AXIS2_PLACEMENT_3D('',#169482,#112580,#112581);
#99161=AXIS2_PLACEMENT_3D('',#169527,#112583,#112584);
#99162=AXIS2_PLACEMENT_3D('',#169575,#112586,#112587);
#99163=AXIS2_PLACEMENT_3D('',#169620,#112589,#112590);
#99164=AXIS2_PLACEMENT_3D('',#169668,#112592,#112593);
#99165=AXIS2_PLACEMENT_3D('',#169713,#112595,#112596);
#99166=AXIS2_PLACEMENT_3D('',#169761,#112598,#112599);
#99167=AXIS2_PLACEMENT_3D('',#169806,#112601,#112602);
#99168=AXIS2_PLACEMENT_3D('',#169854,#112604,#112605);
#99169=AXIS2_PLACEMENT_3D('',#169899,#112607,#112608);
#99170=AXIS2_PLACEMENT_3D('',#169947,#112610,#112611);
#99171=AXIS2_PLACEMENT_3D('',#169992,#112613,#112614);
#99172=AXIS2_PLACEMENT_3D('',#170040,#112616,#112617);
#99173=AXIS2_PLACEMENT_3D('',#170085,#112619,#112620);
#99174=AXIS2_PLACEMENT_3D('',#170133,#112622,#112623);
#99175=AXIS2_PLACEMENT_3D('',#170178,#112625,#112626);
#99176=AXIS2_PLACEMENT_3D('',#170226,#112628,#112629);
#99177=AXIS2_PLACEMENT_3D('',#170271,#112631,#112632);
#99178=AXIS2_PLACEMENT_3D('',#170319,#112634,#112635);
#99179=AXIS2_PLACEMENT_3D('',#170364,#112637,#112638);
#99180=AXIS2_PLACEMENT_3D('',#170412,#112640,#112641);
#99181=AXIS2_PLACEMENT_3D('',#170503,#112645,#112646);
#99182=AXIS2_PLACEMENT_3D('',#170548,#112648,#112649);
#99183=AXIS2_PLACEMENT_3D('',#170596,#112651,#112652);
#99184=AXIS2_PLACEMENT_3D('',#170641,#112654,#112655);
#99185=AXIS2_PLACEMENT_3D('',#170689,#112657,#112658);
#99186=AXIS2_PLACEMENT_3D('',#170734,#112660,#112661);
#99187=AXIS2_PLACEMENT_3D('',#170782,#112663,#112664);
#99188=AXIS2_PLACEMENT_3D('',#170827,#112666,#112667);
#99189=AXIS2_PLACEMENT_3D('',#170875,#112669,#112670);
#99190=AXIS2_PLACEMENT_3D('',#170920,#112672,#112673);
#99191=AXIS2_PLACEMENT_3D('',#170968,#112675,#112676);
#99192=AXIS2_PLACEMENT_3D('',#171013,#112678,#112679);
#99193=AXIS2_PLACEMENT_3D('',#171061,#112681,#112682);
#99194=AXIS2_PLACEMENT_3D('',#171106,#112684,#112685);
#99195=AXIS2_PLACEMENT_3D('',#171154,#112687,#112688);
#99196=AXIS2_PLACEMENT_3D('',#171199,#112690,#112691);
#99197=AXIS2_PLACEMENT_3D('',#171247,#112693,#112694);
#99198=AXIS2_PLACEMENT_3D('',#171292,#112696,#112697);
#99199=AXIS2_PLACEMENT_3D('',#171340,#112699,#112700);
#99200=AXIS2_PLACEMENT_3D('',#171385,#112702,#112703);
#99201=AXIS2_PLACEMENT_3D('',#171433,#112705,#112706);
#99202=AXIS2_PLACEMENT_3D('',#171478,#112708,#112709);
#99203=AXIS2_PLACEMENT_3D('',#171526,#112711,#112712);
#99204=AXIS2_PLACEMENT_3D('',#171571,#112714,#112715);
#99205=AXIS2_PLACEMENT_3D('',#171619,#112717,#112718);
#99206=AXIS2_PLACEMENT_3D('',#171664,#112720,#112721);
#99207=AXIS2_PLACEMENT_3D('',#171712,#112723,#112724);
#99208=AXIS2_PLACEMENT_3D('',#171757,#112726,#112727);
#99209=AXIS2_PLACEMENT_3D('',#171805,#112729,#112730);
#99210=AXIS2_PLACEMENT_3D('',#171895,#112733,#112734);
#99211=AXIS2_PLACEMENT_3D('',#171940,#112736,#112737);
#99212=AXIS2_PLACEMENT_3D('',#171988,#112739,#112740);
#99213=AXIS2_PLACEMENT_3D('',#172033,#112742,#112743);
#99214=AXIS2_PLACEMENT_3D('',#172081,#112745,#112746);
#99215=AXIS2_PLACEMENT_3D('',#172126,#112748,#112749);
#99216=AXIS2_PLACEMENT_3D('',#172174,#112751,#112752);
#99217=AXIS2_PLACEMENT_3D('',#172219,#112754,#112755);
#99218=AXIS2_PLACEMENT_3D('',#172267,#112757,#112758);
#99219=AXIS2_PLACEMENT_3D('',#172312,#112760,#112761);
#99220=AXIS2_PLACEMENT_3D('',#172360,#112763,#112764);
#99221=AXIS2_PLACEMENT_3D('',#172405,#112766,#112767);
#99222=AXIS2_PLACEMENT_3D('',#172453,#112769,#112770);
#99223=AXIS2_PLACEMENT_3D('',#172498,#112772,#112773);
#99224=AXIS2_PLACEMENT_3D('',#172546,#112775,#112776);
#99225=AXIS2_PLACEMENT_3D('',#172591,#112778,#112779);
#99226=AXIS2_PLACEMENT_3D('',#172639,#112781,#112782);
#99227=AXIS2_PLACEMENT_3D('',#172684,#112784,#112785);
#99228=AXIS2_PLACEMENT_3D('',#172732,#112787,#112788);
#99229=AXIS2_PLACEMENT_3D('',#172777,#112790,#112791);
#99230=AXIS2_PLACEMENT_3D('',#172825,#112793,#112794);
#99231=AXIS2_PLACEMENT_3D('',#172870,#112796,#112797);
#99232=AXIS2_PLACEMENT_3D('',#172918,#112799,#112800);
#99233=AXIS2_PLACEMENT_3D('',#172963,#112802,#112803);
#99234=AXIS2_PLACEMENT_3D('',#173011,#112805,#112806);
#99235=AXIS2_PLACEMENT_3D('',#173056,#112808,#112809);
#99236=AXIS2_PLACEMENT_3D('',#173104,#112811,#112812);
#99237=AXIS2_PLACEMENT_3D('',#173149,#112814,#112815);
#99238=AXIS2_PLACEMENT_3D('',#173197,#112817,#112818);
#99239=AXIS2_PLACEMENT_3D('',#173240,#112820,#112821);
#99240=AXIS2_PLACEMENT_3D('',#173282,#112823,#112824);
#99241=AXIS2_PLACEMENT_3D('',#173327,#112826,#112827);
#99242=AXIS2_PLACEMENT_3D('',#173369,#112829,#112830);
#99243=AXIS2_PLACEMENT_3D('',#173414,#112832,#112833);
#99244=AXIS2_PLACEMENT_3D('',#173456,#112835,#112836);
#99245=AXIS2_PLACEMENT_3D('',#173501,#112838,#112839);
#99246=AXIS2_PLACEMENT_3D('',#173543,#112841,#112842);
#99247=AXIS2_PLACEMENT_3D('',#173588,#112844,#112845);
#99248=AXIS2_PLACEMENT_3D('',#173630,#112847,#112848);
#99249=AXIS2_PLACEMENT_3D('',#173675,#112850,#112851);
#99250=AXIS2_PLACEMENT_3D('',#173717,#112853,#112854);
#99251=AXIS2_PLACEMENT_3D('',#173762,#112856,#112857);
#99252=AXIS2_PLACEMENT_3D('',#173804,#112859,#112860);
#99253=AXIS2_PLACEMENT_3D('',#173849,#112862,#112863);
#99254=AXIS2_PLACEMENT_3D('',#173891,#112865,#112866);
#99255=AXIS2_PLACEMENT_3D('',#173936,#112868,#112869);
#99256=AXIS2_PLACEMENT_3D('',#173978,#112871,#112872);
#99257=AXIS2_PLACEMENT_3D('',#174023,#112874,#112875);
#99258=AXIS2_PLACEMENT_3D('',#174065,#112877,#112878);
#99259=AXIS2_PLACEMENT_3D('',#174110,#112880,#112881);
#99260=AXIS2_PLACEMENT_3D('',#174152,#112883,#112884);
#99261=AXIS2_PLACEMENT_3D('',#174197,#112886,#112887);
#99262=AXIS2_PLACEMENT_3D('',#174239,#112889,#112890);
#99263=AXIS2_PLACEMENT_3D('',#174284,#112892,#112893);
#99264=AXIS2_PLACEMENT_3D('',#174326,#112895,#112896);
#99265=AXIS2_PLACEMENT_3D('',#174371,#112898,#112899);
#99266=AXIS2_PLACEMENT_3D('',#174413,#112901,#112902);
#99267=AXIS2_PLACEMENT_3D('',#174458,#112904,#112905);
#99268=AXIS2_PLACEMENT_3D('',#174500,#112907,#112908);
#99269=AXIS2_PLACEMENT_3D('',#174545,#112910,#112911);
#99270=AXIS2_PLACEMENT_3D('',#174587,#112913,#112914);
#99271=AXIS2_PLACEMENT_3D('',#174632,#112916,#112917);
#99272=AXIS2_PLACEMENT_3D('',#174674,#112919,#112920);
#99273=AXIS2_PLACEMENT_3D('',#174719,#112922,#112923);
#99274=AXIS2_PLACEMENT_3D('',#174761,#112925,#112926);
#99275=AXIS2_PLACEMENT_3D('',#174806,#112928,#112929);
#99276=AXIS2_PLACEMENT_3D('',#174848,#112931,#112932);
#99277=AXIS2_PLACEMENT_3D('',#174893,#112934,#112935);
#99278=AXIS2_PLACEMENT_3D('',#174935,#112937,#112938);
#99279=AXIS2_PLACEMENT_3D('',#174980,#112940,#112941);
#99280=AXIS2_PLACEMENT_3D('',#175022,#112943,#112944);
#99281=AXIS2_PLACEMENT_3D('',#175067,#112946,#112947);
#99282=AXIS2_PLACEMENT_3D('',#175109,#112949,#112950);
#99283=AXIS2_PLACEMENT_3D('',#175154,#112952,#112953);
#99284=AXIS2_PLACEMENT_3D('',#175196,#112955,#112956);
#99285=AXIS2_PLACEMENT_3D('',#175241,#112958,#112959);
#99286=AXIS2_PLACEMENT_3D('',#175283,#112961,#112962);
#99287=AXIS2_PLACEMENT_3D('',#175328,#112964,#112965);
#99288=AXIS2_PLACEMENT_3D('',#175370,#112967,#112968);
#99289=AXIS2_PLACEMENT_3D('',#175415,#112970,#112971);
#99290=AXIS2_PLACEMENT_3D('',#175457,#112973,#112974);
#99291=AXIS2_PLACEMENT_3D('',#175502,#112976,#112977);
#99292=AXIS2_PLACEMENT_3D('',#175544,#112979,#112980);
#99293=AXIS2_PLACEMENT_3D('',#175589,#112982,#112983);
#99294=AXIS2_PLACEMENT_3D('',#175631,#112985,#112986);
#99295=AXIS2_PLACEMENT_3D('',#175676,#112988,#112989);
#99296=AXIS2_PLACEMENT_3D('',#175718,#112991,#112992);
#99297=AXIS2_PLACEMENT_3D('',#175763,#112994,#112995);
#99298=AXIS2_PLACEMENT_3D('',#175805,#112997,#112998);
#99299=AXIS2_PLACEMENT_3D('',#175850,#113000,#113001);
#99300=AXIS2_PLACEMENT_3D('',#175853,#113003,#113004);
#99301=AXIS2_PLACEMENT_3D('',#175895,#113006,#113007);
#99302=AXIS2_PLACEMENT_3D('',#175940,#113009,#113010);
#99303=AXIS2_PLACEMENT_3D('',#175982,#113012,#113013);
#99304=AXIS2_PLACEMENT_3D('',#176027,#113015,#113016);
#99305=AXIS2_PLACEMENT_3D('',#176069,#113018,#113019);
#99306=AXIS2_PLACEMENT_3D('',#176114,#113021,#113022);
#99307=AXIS2_PLACEMENT_3D('',#176156,#113024,#113025);
#99308=AXIS2_PLACEMENT_3D('',#176201,#113027,#113028);
#99309=AXIS2_PLACEMENT_3D('',#176243,#113030,#113031);
#99310=AXIS2_PLACEMENT_3D('',#176288,#113033,#113034);
#99311=AXIS2_PLACEMENT_3D('',#176330,#113036,#113037);
#99312=AXIS2_PLACEMENT_3D('',#176375,#113039,#113040);
#99313=AXIS2_PLACEMENT_3D('',#176417,#113042,#113043);
#99314=AXIS2_PLACEMENT_3D('',#176462,#113045,#113046);
#99315=AXIS2_PLACEMENT_3D('',#176504,#113048,#113049);
#99316=AXIS2_PLACEMENT_3D('',#176549,#113051,#113052);
#99317=AXIS2_PLACEMENT_3D('',#176591,#113054,#113055);
#99318=AXIS2_PLACEMENT_3D('',#176636,#113057,#113058);
#99319=AXIS2_PLACEMENT_3D('',#176678,#113060,#113061);
#99320=AXIS2_PLACEMENT_3D('',#176723,#113063,#113064);
#99321=AXIS2_PLACEMENT_3D('',#176765,#113066,#113067);
#99322=AXIS2_PLACEMENT_3D('',#176810,#113069,#113070);
#99323=AXIS2_PLACEMENT_3D('',#176852,#113072,#113073);
#99324=AXIS2_PLACEMENT_3D('',#176897,#113075,#113076);
#99325=AXIS2_PLACEMENT_3D('',#176939,#113078,#113079);
#99326=AXIS2_PLACEMENT_3D('',#176984,#113081,#113082);
#99327=AXIS2_PLACEMENT_3D('',#177026,#113084,#113085);
#99328=AXIS2_PLACEMENT_3D('',#177071,#113087,#113088);
#99329=AXIS2_PLACEMENT_3D('',#177113,#113090,#113091);
#99330=AXIS2_PLACEMENT_3D('',#177197,#113094,#113095);
#99331=AXIS2_PLACEMENT_3D('',#177242,#113097,#113098);
#99332=AXIS2_PLACEMENT_3D('',#177284,#113100,#113101);
#99333=AXIS2_PLACEMENT_3D('',#177329,#113103,#113104);
#99334=AXIS2_PLACEMENT_3D('',#177371,#113106,#113107);
#99335=AXIS2_PLACEMENT_3D('',#177416,#113109,#113110);
#99336=AXIS2_PLACEMENT_3D('',#177458,#113112,#113113);
#99337=AXIS2_PLACEMENT_3D('',#177503,#113115,#113116);
#99338=AXIS2_PLACEMENT_3D('',#177545,#113118,#113119);
#99339=AXIS2_PLACEMENT_3D('',#177590,#113121,#113122);
#99340=AXIS2_PLACEMENT_3D('',#177632,#113124,#113125);
#99341=AXIS2_PLACEMENT_3D('',#177677,#113127,#113128);
#99342=AXIS2_PLACEMENT_3D('',#177719,#113130,#113131);
#99343=AXIS2_PLACEMENT_3D('',#177764,#113133,#113134);
#99344=AXIS2_PLACEMENT_3D('',#177806,#113136,#113137);
#99345=AXIS2_PLACEMENT_3D('',#177851,#113139,#113140);
#99346=AXIS2_PLACEMENT_3D('',#177893,#113142,#113143);
#99347=AXIS2_PLACEMENT_3D('',#177938,#113145,#113146);
#99348=AXIS2_PLACEMENT_3D('',#177980,#113148,#113149);
#99349=AXIS2_PLACEMENT_3D('',#178025,#113151,#113152);
#99350=AXIS2_PLACEMENT_3D('',#178067,#113154,#113155);
#99351=AXIS2_PLACEMENT_3D('',#178112,#113157,#113158);
#99352=AXIS2_PLACEMENT_3D('',#178154,#113160,#113161);
#99353=AXIS2_PLACEMENT_3D('',#178199,#113163,#113164);
#99354=AXIS2_PLACEMENT_3D('',#178241,#113166,#113167);
#99355=AXIS2_PLACEMENT_3D('',#178286,#113169,#113170);
#99356=AXIS2_PLACEMENT_3D('',#178328,#113172,#113173);
#99357=AXIS2_PLACEMENT_3D('',#178373,#113175,#113176);
#99358=AXIS2_PLACEMENT_3D('',#178415,#113178,#113179);
#99359=AXIS2_PLACEMENT_3D('',#178458,#113181,#113182);
#99360=AXIS2_PLACEMENT_3D('',#178461,#113183,#113184);
#99361=AXIS2_PLACEMENT_3D('',#178463,#113186,#113187);
#99362=AXIS2_PLACEMENT_3D('',#178464,#113188,#113189);
#99363=AXIS2_PLACEMENT_3D('',#178467,#113191,#113192);
#99364=AXIS2_PLACEMENT_3D('',#178468,#113193,#113194);
#99365=AXIS2_PLACEMENT_3D('',#178471,#113195,#113196);
#99366=AXIS2_PLACEMENT_3D('',#178475,#113198,#113199);
#99367=AXIS2_PLACEMENT_3D('',#178479,#113201,#113202);
#99368=AXIS2_PLACEMENT_3D('',#178480,#113203,#113204);
#99369=AXIS2_PLACEMENT_3D('',#178481,#113205,#113206);
#99370=AXIS2_PLACEMENT_3D('',#178484,#113207,#113208);
#99371=AXIS2_PLACEMENT_3D('',#178487,#113211,#113212);
#99372=AXIS2_PLACEMENT_3D('',#178490,#113213,#113214);
#99373=AXIS2_PLACEMENT_3D('',#178494,#113216,#113217);
#99374=AXIS2_PLACEMENT_3D('',#178496,#113219,#113220);
#99375=AXIS2_PLACEMENT_3D('',#178499,#113221,#113222);
#99376=AXIS2_PLACEMENT_3D('',#178503,#113224,#113225);
#99377=AXIS2_PLACEMENT_3D('',#178507,#113227,#113228);
#99378=AXIS2_PLACEMENT_3D('',#178508,#113229,#113230);
#99379=AXIS2_PLACEMENT_3D('',#178509,#113231,#113232);
#99380=AXIS2_PLACEMENT_3D('',#178512,#113233,#113234);
#99381=AXIS2_PLACEMENT_3D('',#178515,#113237,#113238);
#99382=AXIS2_PLACEMENT_3D('',#178516,#113239,#113240);
#99383=AXIS2_PLACEMENT_3D('',#178517,#113241,#113242);
#99384=AXIS2_PLACEMENT_3D('',#178518,#113243,#113244);
#99385=AXIS2_PLACEMENT_3D('',#178519,#113245,#113246);
#99386=AXIS2_PLACEMENT_3D('',#178520,#113247,#113248);
#99387=AXIS2_PLACEMENT_3D('',#178521,#113249,#113250);
#99388=AXIS2_PLACEMENT_3D('',#178522,#113251,#113252);
#99389=AXIS2_PLACEMENT_3D('',#178523,#113253,#113254);
#99390=AXIS2_PLACEMENT_3D('',#178524,#113255,#113256);
#99391=AXIS2_PLACEMENT_3D('',#178525,#113257,#113258);
#99392=AXIS2_PLACEMENT_3D('',#178526,#113259,#113260);
#99393=AXIS2_PLACEMENT_3D('',#178527,#113261,#113262);
#99394=AXIS2_PLACEMENT_3D('',#178530,#113263,#113264);
#99395=AXIS2_PLACEMENT_3D('',#178534,#113266,#113267);
#99396=AXIS2_PLACEMENT_3D('',#178536,#113268,#113269);
#99397=AXIS2_PLACEMENT_3D('',#178538,#113270,#113271);
#99398=AXIS2_PLACEMENT_3D('',#178540,#113273,#113274);
#99399=AXIS2_PLACEMENT_3D('',#178544,#113276,#113277);
#99400=AXIS2_PLACEMENT_3D('',#178546,#113279,#113280);
#99401=AXIS2_PLACEMENT_3D('',#178549,#113281,#113282);
#99402=AXIS2_PLACEMENT_3D('',#178553,#113284,#113285);
#99403=AXIS2_PLACEMENT_3D('',#178555,#113287,#113288);
#99404=AXIS2_PLACEMENT_3D('',#178558,#113289,#113290);
#99405=AXIS2_PLACEMENT_3D('',#178562,#113292,#113293);
#99406=AXIS2_PLACEMENT_3D('',#178564,#113294,#113295);
#99407=AXIS2_PLACEMENT_3D('',#178566,#113296,#113297);
#99408=AXIS2_PLACEMENT_3D('',#178568,#113299,#113300);
#99409=AXIS2_PLACEMENT_3D('',#178572,#113302,#113303);
#99410=AXIS2_PLACEMENT_3D('',#178574,#113305,#113306);
#99411=AXIS2_PLACEMENT_3D('',#178575,#113307,#113308);
#99412=AXIS2_PLACEMENT_3D('',#178576,#113309,#113310);
#99413=AXIS2_PLACEMENT_3D('',#178577,#113311,#113312);
#99414=AXIS2_PLACEMENT_3D('',#178578,#113313,#113314);
#99415=AXIS2_PLACEMENT_3D('',#178579,#113315,#113316);
#99416=AXIS2_PLACEMENT_3D('',#178580,#113317,#113318);
#99417=AXIS2_PLACEMENT_3D('',#178581,#113319,#113320);
#99418=AXIS2_PLACEMENT_3D('',#178582,#113321,#113322);
#99419=AXIS2_PLACEMENT_3D('',#178583,#113323,#113324);
#99420=AXIS2_PLACEMENT_3D('',#178584,#113325,#113326);
#99421=AXIS2_PLACEMENT_3D('',#178585,#113327,#113328);
#99422=AXIS2_PLACEMENT_3D('',#178586,#113329,#113330);
#99423=AXIS2_PLACEMENT_3D('',#178589,#113331,#113332);
#99424=AXIS2_PLACEMENT_3D('',#178593,#113334,#113335);
#99425=AXIS2_PLACEMENT_3D('',#178595,#113336,#113337);
#99426=AXIS2_PLACEMENT_3D('',#178597,#113338,#113339);
#99427=AXIS2_PLACEMENT_3D('',#178599,#113341,#113342);
#99428=AXIS2_PLACEMENT_3D('',#178603,#113344,#113345);
#99429=AXIS2_PLACEMENT_3D('',#178605,#113347,#113348);
#99430=AXIS2_PLACEMENT_3D('',#178608,#113349,#113350);
#99431=AXIS2_PLACEMENT_3D('',#178612,#113352,#113353);
#99432=AXIS2_PLACEMENT_3D('',#178614,#113355,#113356);
#99433=AXIS2_PLACEMENT_3D('',#178617,#113357,#113358);
#99434=AXIS2_PLACEMENT_3D('',#178621,#113360,#113361);
#99435=AXIS2_PLACEMENT_3D('',#178623,#113362,#113363);
#99436=AXIS2_PLACEMENT_3D('',#178625,#113364,#113365);
#99437=AXIS2_PLACEMENT_3D('',#178627,#113367,#113368);
#99438=AXIS2_PLACEMENT_3D('',#178631,#113370,#113371);
#99439=AXIS2_PLACEMENT_3D('',#178633,#113373,#113374);
#99440=AXIS2_PLACEMENT_3D('',#178634,#113375,#113376);
#99441=AXIS2_PLACEMENT_3D('',#178635,#113377,#113378);
#99442=AXIS2_PLACEMENT_3D('',#178636,#113379,#113380);
#99443=AXIS2_PLACEMENT_3D('',#178637,#113381,#113382);
#99444=AXIS2_PLACEMENT_3D('',#178638,#113383,#113384);
#99445=AXIS2_PLACEMENT_3D('',#178639,#113385,#113386);
#99446=AXIS2_PLACEMENT_3D('',#178640,#113387,#113388);
#99447=AXIS2_PLACEMENT_3D('',#178641,#113389,#113390);
#99448=AXIS2_PLACEMENT_3D('',#178642,#113391,#113392);
#99449=AXIS2_PLACEMENT_3D('',#178643,#113393,#113394);
#99450=AXIS2_PLACEMENT_3D('',#178644,#113395,#113396);
#99451=AXIS2_PLACEMENT_3D('',#178645,#113397,#113398);
#99452=AXIS2_PLACEMENT_3D('',#178648,#113399,#113400);
#99453=AXIS2_PLACEMENT_3D('',#178652,#113402,#113403);
#99454=AXIS2_PLACEMENT_3D('',#178654,#113404,#113405);
#99455=AXIS2_PLACEMENT_3D('',#178656,#113406,#113407);
#99456=AXIS2_PLACEMENT_3D('',#178658,#113409,#113410);
#99457=AXIS2_PLACEMENT_3D('',#178662,#113412,#113413);
#99458=AXIS2_PLACEMENT_3D('',#178664,#113415,#113416);
#99459=AXIS2_PLACEMENT_3D('',#178667,#113417,#113418);
#99460=AXIS2_PLACEMENT_3D('',#178671,#113420,#113421);
#99461=AXIS2_PLACEMENT_3D('',#178673,#113423,#113424);
#99462=AXIS2_PLACEMENT_3D('',#178676,#113425,#113426);
#99463=AXIS2_PLACEMENT_3D('',#178680,#113428,#113429);
#99464=AXIS2_PLACEMENT_3D('',#178682,#113430,#113431);
#99465=AXIS2_PLACEMENT_3D('',#178684,#113432,#113433);
#99466=AXIS2_PLACEMENT_3D('',#178686,#113435,#113436);
#99467=AXIS2_PLACEMENT_3D('',#178690,#113438,#113439);
#99468=AXIS2_PLACEMENT_3D('',#178692,#113441,#113442);
#99469=AXIS2_PLACEMENT_3D('',#178693,#113443,#113444);
#99470=AXIS2_PLACEMENT_3D('',#178694,#113445,#113446);
#99471=AXIS2_PLACEMENT_3D('',#178695,#113447,#113448);
#99472=AXIS2_PLACEMENT_3D('',#178696,#113449,#113450);
#99473=AXIS2_PLACEMENT_3D('',#178697,#113451,#113452);
#99474=AXIS2_PLACEMENT_3D('',#178698,#113453,#113454);
#99475=AXIS2_PLACEMENT_3D('',#178699,#113455,#113456);
#99476=AXIS2_PLACEMENT_3D('',#178700,#113457,#113458);
#99477=AXIS2_PLACEMENT_3D('',#178701,#113459,#113460);
#99478=AXIS2_PLACEMENT_3D('',#178702,#113461,#113462);
#99479=AXIS2_PLACEMENT_3D('',#178703,#113463,#113464);
#99480=AXIS2_PLACEMENT_3D('',#178704,#113465,#113466);
#99481=AXIS2_PLACEMENT_3D('',#178707,#113467,#113468);
#99482=AXIS2_PLACEMENT_3D('',#178711,#113470,#113471);
#99483=AXIS2_PLACEMENT_3D('',#178713,#113472,#113473);
#99484=AXIS2_PLACEMENT_3D('',#178715,#113474,#113475);
#99485=AXIS2_PLACEMENT_3D('',#178717,#113477,#113478);
#99486=AXIS2_PLACEMENT_3D('',#178721,#113480,#113481);
#99487=AXIS2_PLACEMENT_3D('',#178723,#113483,#113484);
#99488=AXIS2_PLACEMENT_3D('',#178726,#113485,#113486);
#99489=AXIS2_PLACEMENT_3D('',#178730,#113488,#113489);
#99490=AXIS2_PLACEMENT_3D('',#178732,#113491,#113492);
#99491=AXIS2_PLACEMENT_3D('',#178735,#113493,#113494);
#99492=AXIS2_PLACEMENT_3D('',#178739,#113496,#113497);
#99493=AXIS2_PLACEMENT_3D('',#178741,#113498,#113499);
#99494=AXIS2_PLACEMENT_3D('',#178743,#113500,#113501);
#99495=AXIS2_PLACEMENT_3D('',#178745,#113503,#113504);
#99496=AXIS2_PLACEMENT_3D('',#178749,#113506,#113507);
#99497=AXIS2_PLACEMENT_3D('',#178751,#113509,#113510);
#99498=AXIS2_PLACEMENT_3D('',#178752,#113511,#113512);
#99499=AXIS2_PLACEMENT_3D('',#178753,#113513,#113514);
#99500=AXIS2_PLACEMENT_3D('',#178754,#113515,#113516);
#99501=AXIS2_PLACEMENT_3D('',#178755,#113517,#113518);
#99502=AXIS2_PLACEMENT_3D('',#178756,#113519,#113520);
#99503=AXIS2_PLACEMENT_3D('',#178757,#113521,#113522);
#99504=AXIS2_PLACEMENT_3D('',#178758,#113523,#113524);
#99505=AXIS2_PLACEMENT_3D('',#178759,#113525,#113526);
#99506=AXIS2_PLACEMENT_3D('',#178760,#113527,#113528);
#99507=AXIS2_PLACEMENT_3D('',#178761,#113529,#113530);
#99508=AXIS2_PLACEMENT_3D('',#178762,#113531,#113532);
#99509=AXIS2_PLACEMENT_3D('',#178763,#113533,#113534);
#99510=AXIS2_PLACEMENT_3D('',#178766,#113535,#113536);
#99511=AXIS2_PLACEMENT_3D('',#178770,#113538,#113539);
#99512=AXIS2_PLACEMENT_3D('',#178772,#113540,#113541);
#99513=AXIS2_PLACEMENT_3D('',#178774,#113542,#113543);
#99514=AXIS2_PLACEMENT_3D('',#178776,#113545,#113546);
#99515=AXIS2_PLACEMENT_3D('',#178780,#113548,#113549);
#99516=AXIS2_PLACEMENT_3D('',#178782,#113551,#113552);
#99517=AXIS2_PLACEMENT_3D('',#178785,#113553,#113554);
#99518=AXIS2_PLACEMENT_3D('',#178789,#113556,#113557);
#99519=AXIS2_PLACEMENT_3D('',#178791,#113559,#113560);
#99520=AXIS2_PLACEMENT_3D('',#178794,#113561,#113562);
#99521=AXIS2_PLACEMENT_3D('',#178798,#113564,#113565);
#99522=AXIS2_PLACEMENT_3D('',#178800,#113566,#113567);
#99523=AXIS2_PLACEMENT_3D('',#178802,#113568,#113569);
#99524=AXIS2_PLACEMENT_3D('',#178804,#113571,#113572);
#99525=AXIS2_PLACEMENT_3D('',#178808,#113574,#113575);
#99526=AXIS2_PLACEMENT_3D('',#178810,#113577,#113578);
#99527=AXIS2_PLACEMENT_3D('',#178811,#113579,#113580);
#99528=AXIS2_PLACEMENT_3D('',#178812,#113581,#113582);
#99529=AXIS2_PLACEMENT_3D('',#178813,#113583,#113584);
#99530=AXIS2_PLACEMENT_3D('',#178814,#113585,#113586);
#99531=AXIS2_PLACEMENT_3D('',#178815,#113587,#113588);
#99532=AXIS2_PLACEMENT_3D('',#178816,#113589,#113590);
#99533=AXIS2_PLACEMENT_3D('',#178817,#113591,#113592);
#99534=AXIS2_PLACEMENT_3D('',#178818,#113593,#113594);
#99535=AXIS2_PLACEMENT_3D('',#178819,#113595,#113596);
#99536=AXIS2_PLACEMENT_3D('',#178820,#113597,#113598);
#99537=AXIS2_PLACEMENT_3D('',#178821,#113599,#113600);
#99538=AXIS2_PLACEMENT_3D('',#178822,#113601,#113602);
#99539=AXIS2_PLACEMENT_3D('',#178825,#113603,#113604);
#99540=AXIS2_PLACEMENT_3D('',#178829,#113606,#113607);
#99541=AXIS2_PLACEMENT_3D('',#178831,#113608,#113609);
#99542=AXIS2_PLACEMENT_3D('',#178833,#113610,#113611);
#99543=AXIS2_PLACEMENT_3D('',#178835,#113613,#113614);
#99544=AXIS2_PLACEMENT_3D('',#178839,#113616,#113617);
#99545=AXIS2_PLACEMENT_3D('',#178841,#113619,#113620);
#99546=AXIS2_PLACEMENT_3D('',#178844,#113621,#113622);
#99547=AXIS2_PLACEMENT_3D('',#178848,#113624,#113625);
#99548=AXIS2_PLACEMENT_3D('',#178850,#113627,#113628);
#99549=AXIS2_PLACEMENT_3D('',#178853,#113629,#113630);
#99550=AXIS2_PLACEMENT_3D('',#178857,#113632,#113633);
#99551=AXIS2_PLACEMENT_3D('',#178859,#113634,#113635);
#99552=AXIS2_PLACEMENT_3D('',#178861,#113636,#113637);
#99553=AXIS2_PLACEMENT_3D('',#178863,#113639,#113640);
#99554=AXIS2_PLACEMENT_3D('',#178867,#113642,#113643);
#99555=AXIS2_PLACEMENT_3D('',#178869,#113645,#113646);
#99556=AXIS2_PLACEMENT_3D('',#178870,#113647,#113648);
#99557=AXIS2_PLACEMENT_3D('',#178871,#113649,#113650);
#99558=AXIS2_PLACEMENT_3D('',#178872,#113651,#113652);
#99559=AXIS2_PLACEMENT_3D('',#178873,#113653,#113654);
#99560=AXIS2_PLACEMENT_3D('',#178874,#113655,#113656);
#99561=AXIS2_PLACEMENT_3D('',#178875,#113657,#113658);
#99562=AXIS2_PLACEMENT_3D('',#178876,#113659,#113660);
#99563=AXIS2_PLACEMENT_3D('',#178877,#113661,#113662);
#99564=AXIS2_PLACEMENT_3D('',#178878,#113663,#113664);
#99565=AXIS2_PLACEMENT_3D('',#178879,#113665,#113666);
#99566=AXIS2_PLACEMENT_3D('',#178880,#113667,#113668);
#99567=AXIS2_PLACEMENT_3D('',#178881,#113669,#113670);
#99568=AXIS2_PLACEMENT_3D('',#178884,#113671,#113672);
#99569=AXIS2_PLACEMENT_3D('',#178888,#113674,#113675);
#99570=AXIS2_PLACEMENT_3D('',#178890,#113676,#113677);
#99571=AXIS2_PLACEMENT_3D('',#178892,#113678,#113679);
#99572=AXIS2_PLACEMENT_3D('',#178894,#113681,#113682);
#99573=AXIS2_PLACEMENT_3D('',#178898,#113684,#113685);
#99574=AXIS2_PLACEMENT_3D('',#178900,#113687,#113688);
#99575=AXIS2_PLACEMENT_3D('',#178903,#113689,#113690);
#99576=AXIS2_PLACEMENT_3D('',#178907,#113692,#113693);
#99577=AXIS2_PLACEMENT_3D('',#178909,#113695,#113696);
#99578=AXIS2_PLACEMENT_3D('',#178912,#113697,#113698);
#99579=AXIS2_PLACEMENT_3D('',#178916,#113700,#113701);
#99580=AXIS2_PLACEMENT_3D('',#178918,#113702,#113703);
#99581=AXIS2_PLACEMENT_3D('',#178920,#113704,#113705);
#99582=AXIS2_PLACEMENT_3D('',#178922,#113707,#113708);
#99583=AXIS2_PLACEMENT_3D('',#178926,#113710,#113711);
#99584=AXIS2_PLACEMENT_3D('',#178928,#113713,#113714);
#99585=AXIS2_PLACEMENT_3D('',#178929,#113715,#113716);
#99586=AXIS2_PLACEMENT_3D('',#178930,#113717,#113718);
#99587=AXIS2_PLACEMENT_3D('',#178931,#113719,#113720);
#99588=AXIS2_PLACEMENT_3D('',#178932,#113721,#113722);
#99589=AXIS2_PLACEMENT_3D('',#178933,#113723,#113724);
#99590=AXIS2_PLACEMENT_3D('',#178934,#113725,#113726);
#99591=AXIS2_PLACEMENT_3D('',#178935,#113727,#113728);
#99592=AXIS2_PLACEMENT_3D('',#178936,#113729,#113730);
#99593=AXIS2_PLACEMENT_3D('',#178937,#113731,#113732);
#99594=AXIS2_PLACEMENT_3D('',#178938,#113733,#113734);
#99595=AXIS2_PLACEMENT_3D('',#178939,#113735,#113736);
#99596=AXIS2_PLACEMENT_3D('',#178940,#113737,#113738);
#99597=AXIS2_PLACEMENT_3D('',#178943,#113739,#113740);
#99598=AXIS2_PLACEMENT_3D('',#178947,#113742,#113743);
#99599=AXIS2_PLACEMENT_3D('',#178949,#113744,#113745);
#99600=AXIS2_PLACEMENT_3D('',#178951,#113746,#113747);
#99601=AXIS2_PLACEMENT_3D('',#178953,#113749,#113750);
#99602=AXIS2_PLACEMENT_3D('',#178957,#113752,#113753);
#99603=AXIS2_PLACEMENT_3D('',#178959,#113755,#113756);
#99604=AXIS2_PLACEMENT_3D('',#178962,#113757,#113758);
#99605=AXIS2_PLACEMENT_3D('',#178966,#113760,#113761);
#99606=AXIS2_PLACEMENT_3D('',#178968,#113763,#113764);
#99607=AXIS2_PLACEMENT_3D('',#178971,#113765,#113766);
#99608=AXIS2_PLACEMENT_3D('',#178975,#113768,#113769);
#99609=AXIS2_PLACEMENT_3D('',#178977,#113770,#113771);
#99610=AXIS2_PLACEMENT_3D('',#178979,#113772,#113773);
#99611=AXIS2_PLACEMENT_3D('',#178981,#113775,#113776);
#99612=AXIS2_PLACEMENT_3D('',#178985,#113778,#113779);
#99613=AXIS2_PLACEMENT_3D('',#178987,#113781,#113782);
#99614=AXIS2_PLACEMENT_3D('',#178988,#113783,#113784);
#99615=AXIS2_PLACEMENT_3D('',#178989,#113785,#113786);
#99616=AXIS2_PLACEMENT_3D('',#178990,#113787,#113788);
#99617=AXIS2_PLACEMENT_3D('',#178991,#113789,#113790);
#99618=AXIS2_PLACEMENT_3D('',#178992,#113791,#113792);
#99619=AXIS2_PLACEMENT_3D('',#178993,#113793,#113794);
#99620=AXIS2_PLACEMENT_3D('',#178994,#113795,#113796);
#99621=AXIS2_PLACEMENT_3D('',#178995,#113797,#113798);
#99622=AXIS2_PLACEMENT_3D('',#178996,#113799,#113800);
#99623=AXIS2_PLACEMENT_3D('',#178997,#113801,#113802);
#99624=AXIS2_PLACEMENT_3D('',#178998,#113803,#113804);
#99625=AXIS2_PLACEMENT_3D('',#178999,#113805,#113806);
#99626=AXIS2_PLACEMENT_3D('',#179002,#113807,#113808);
#99627=AXIS2_PLACEMENT_3D('',#179006,#113810,#113811);
#99628=AXIS2_PLACEMENT_3D('',#179008,#113812,#113813);
#99629=AXIS2_PLACEMENT_3D('',#179010,#113814,#113815);
#99630=AXIS2_PLACEMENT_3D('',#179012,#113817,#113818);
#99631=AXIS2_PLACEMENT_3D('',#179016,#113820,#113821);
#99632=AXIS2_PLACEMENT_3D('',#179018,#113823,#113824);
#99633=AXIS2_PLACEMENT_3D('',#179021,#113825,#113826);
#99634=AXIS2_PLACEMENT_3D('',#179025,#113828,#113829);
#99635=AXIS2_PLACEMENT_3D('',#179027,#113831,#113832);
#99636=AXIS2_PLACEMENT_3D('',#179030,#113833,#113834);
#99637=AXIS2_PLACEMENT_3D('',#179034,#113836,#113837);
#99638=AXIS2_PLACEMENT_3D('',#179036,#113838,#113839);
#99639=AXIS2_PLACEMENT_3D('',#179038,#113840,#113841);
#99640=AXIS2_PLACEMENT_3D('',#179040,#113843,#113844);
#99641=AXIS2_PLACEMENT_3D('',#179044,#113846,#113847);
#99642=AXIS2_PLACEMENT_3D('',#179046,#113849,#113850);
#99643=AXIS2_PLACEMENT_3D('',#179047,#113851,#113852);
#99644=AXIS2_PLACEMENT_3D('',#179048,#113853,#113854);
#99645=AXIS2_PLACEMENT_3D('',#179049,#113855,#113856);
#99646=AXIS2_PLACEMENT_3D('',#179050,#113857,#113858);
#99647=AXIS2_PLACEMENT_3D('',#179051,#113859,#113860);
#99648=AXIS2_PLACEMENT_3D('',#179052,#113861,#113862);
#99649=AXIS2_PLACEMENT_3D('',#179053,#113863,#113864);
#99650=AXIS2_PLACEMENT_3D('',#179054,#113865,#113866);
#99651=AXIS2_PLACEMENT_3D('',#179055,#113867,#113868);
#99652=AXIS2_PLACEMENT_3D('',#179056,#113869,#113870);
#99653=AXIS2_PLACEMENT_3D('',#179057,#113871,#113872);
#99654=AXIS2_PLACEMENT_3D('',#179058,#113873,#113874);
#99655=AXIS2_PLACEMENT_3D('',#179061,#113875,#113876);
#99656=AXIS2_PLACEMENT_3D('',#179065,#113878,#113879);
#99657=AXIS2_PLACEMENT_3D('',#179067,#113880,#113881);
#99658=AXIS2_PLACEMENT_3D('',#179069,#113882,#113883);
#99659=AXIS2_PLACEMENT_3D('',#179071,#113885,#113886);
#99660=AXIS2_PLACEMENT_3D('',#179075,#113888,#113889);
#99661=AXIS2_PLACEMENT_3D('',#179077,#113891,#113892);
#99662=AXIS2_PLACEMENT_3D('',#179080,#113893,#113894);
#99663=AXIS2_PLACEMENT_3D('',#179084,#113896,#113897);
#99664=AXIS2_PLACEMENT_3D('',#179086,#113899,#113900);
#99665=AXIS2_PLACEMENT_3D('',#179089,#113901,#113902);
#99666=AXIS2_PLACEMENT_3D('',#179093,#113904,#113905);
#99667=AXIS2_PLACEMENT_3D('',#179095,#113906,#113907);
#99668=AXIS2_PLACEMENT_3D('',#179097,#113908,#113909);
#99669=AXIS2_PLACEMENT_3D('',#179099,#113911,#113912);
#99670=AXIS2_PLACEMENT_3D('',#179103,#113914,#113915);
#99671=AXIS2_PLACEMENT_3D('',#179105,#113917,#113918);
#99672=AXIS2_PLACEMENT_3D('',#179106,#113919,#113920);
#99673=AXIS2_PLACEMENT_3D('',#179107,#113921,#113922);
#99674=AXIS2_PLACEMENT_3D('',#179108,#113923,#113924);
#99675=AXIS2_PLACEMENT_3D('',#179109,#113925,#113926);
#99676=AXIS2_PLACEMENT_3D('',#179110,#113927,#113928);
#99677=AXIS2_PLACEMENT_3D('',#179111,#113929,#113930);
#99678=AXIS2_PLACEMENT_3D('',#179112,#113931,#113932);
#99679=AXIS2_PLACEMENT_3D('',#179113,#113933,#113934);
#99680=AXIS2_PLACEMENT_3D('',#179114,#113935,#113936);
#99681=AXIS2_PLACEMENT_3D('',#179115,#113937,#113938);
#99682=AXIS2_PLACEMENT_3D('',#179116,#113939,#113940);
#99683=AXIS2_PLACEMENT_3D('',#179117,#113941,#113942);
#99684=AXIS2_PLACEMENT_3D('',#179120,#113943,#113944);
#99685=AXIS2_PLACEMENT_3D('',#179124,#113946,#113947);
#99686=AXIS2_PLACEMENT_3D('',#179126,#113948,#113949);
#99687=AXIS2_PLACEMENT_3D('',#179128,#113950,#113951);
#99688=AXIS2_PLACEMENT_3D('',#179130,#113953,#113954);
#99689=AXIS2_PLACEMENT_3D('',#179134,#113956,#113957);
#99690=AXIS2_PLACEMENT_3D('',#179136,#113959,#113960);
#99691=AXIS2_PLACEMENT_3D('',#179139,#113961,#113962);
#99692=AXIS2_PLACEMENT_3D('',#179143,#113964,#113965);
#99693=AXIS2_PLACEMENT_3D('',#179145,#113967,#113968);
#99694=AXIS2_PLACEMENT_3D('',#179148,#113969,#113970);
#99695=AXIS2_PLACEMENT_3D('',#179152,#113972,#113973);
#99696=AXIS2_PLACEMENT_3D('',#179154,#113974,#113975);
#99697=AXIS2_PLACEMENT_3D('',#179156,#113976,#113977);
#99698=AXIS2_PLACEMENT_3D('',#179158,#113979,#113980);
#99699=AXIS2_PLACEMENT_3D('',#179162,#113982,#113983);
#99700=AXIS2_PLACEMENT_3D('',#179164,#113985,#113986);
#99701=AXIS2_PLACEMENT_3D('',#179165,#113987,#113988);
#99702=AXIS2_PLACEMENT_3D('',#179166,#113989,#113990);
#99703=AXIS2_PLACEMENT_3D('',#179167,#113991,#113992);
#99704=AXIS2_PLACEMENT_3D('',#179168,#113993,#113994);
#99705=AXIS2_PLACEMENT_3D('',#179169,#113995,#113996);
#99706=AXIS2_PLACEMENT_3D('',#179170,#113997,#113998);
#99707=AXIS2_PLACEMENT_3D('',#179171,#113999,#114000);
#99708=AXIS2_PLACEMENT_3D('',#179172,#114001,#114002);
#99709=AXIS2_PLACEMENT_3D('',#179173,#114003,#114004);
#99710=AXIS2_PLACEMENT_3D('',#179174,#114005,#114006);
#99711=AXIS2_PLACEMENT_3D('',#179175,#114007,#114008);
#99712=AXIS2_PLACEMENT_3D('',#179176,#114009,#114010);
#99713=AXIS2_PLACEMENT_3D('',#179179,#114011,#114012);
#99714=AXIS2_PLACEMENT_3D('',#179183,#114014,#114015);
#99715=AXIS2_PLACEMENT_3D('',#179185,#114016,#114017);
#99716=AXIS2_PLACEMENT_3D('',#179187,#114018,#114019);
#99717=AXIS2_PLACEMENT_3D('',#179189,#114021,#114022);
#99718=AXIS2_PLACEMENT_3D('',#179193,#114024,#114025);
#99719=AXIS2_PLACEMENT_3D('',#179195,#114027,#114028);
#99720=AXIS2_PLACEMENT_3D('',#179198,#114029,#114030);
#99721=AXIS2_PLACEMENT_3D('',#179202,#114032,#114033);
#99722=AXIS2_PLACEMENT_3D('',#179204,#114035,#114036);
#99723=AXIS2_PLACEMENT_3D('',#179207,#114037,#114038);
#99724=AXIS2_PLACEMENT_3D('',#179211,#114040,#114041);
#99725=AXIS2_PLACEMENT_3D('',#179213,#114042,#114043);
#99726=AXIS2_PLACEMENT_3D('',#179215,#114044,#114045);
#99727=AXIS2_PLACEMENT_3D('',#179217,#114047,#114048);
#99728=AXIS2_PLACEMENT_3D('',#179221,#114050,#114051);
#99729=AXIS2_PLACEMENT_3D('',#179223,#114053,#114054);
#99730=AXIS2_PLACEMENT_3D('',#179224,#114055,#114056);
#99731=AXIS2_PLACEMENT_3D('',#179225,#114057,#114058);
#99732=AXIS2_PLACEMENT_3D('',#179226,#114059,#114060);
#99733=AXIS2_PLACEMENT_3D('',#179227,#114061,#114062);
#99734=AXIS2_PLACEMENT_3D('',#179228,#114063,#114064);
#99735=AXIS2_PLACEMENT_3D('',#179229,#114065,#114066);
#99736=AXIS2_PLACEMENT_3D('',#179230,#114067,#114068);
#99737=AXIS2_PLACEMENT_3D('',#179231,#114069,#114070);
#99738=AXIS2_PLACEMENT_3D('',#179232,#114071,#114072);
#99739=AXIS2_PLACEMENT_3D('',#179233,#114073,#114074);
#99740=AXIS2_PLACEMENT_3D('',#179234,#114075,#114076);
#99741=AXIS2_PLACEMENT_3D('',#179235,#114077,#114078);
#99742=AXIS2_PLACEMENT_3D('',#179238,#114079,#114080);
#99743=AXIS2_PLACEMENT_3D('',#179242,#114082,#114083);
#99744=AXIS2_PLACEMENT_3D('',#179244,#114084,#114085);
#99745=AXIS2_PLACEMENT_3D('',#179246,#114086,#114087);
#99746=AXIS2_PLACEMENT_3D('',#179248,#114089,#114090);
#99747=AXIS2_PLACEMENT_3D('',#179252,#114092,#114093);
#99748=AXIS2_PLACEMENT_3D('',#179254,#114095,#114096);
#99749=AXIS2_PLACEMENT_3D('',#179257,#114097,#114098);
#99750=AXIS2_PLACEMENT_3D('',#179261,#114100,#114101);
#99751=AXIS2_PLACEMENT_3D('',#179263,#114103,#114104);
#99752=AXIS2_PLACEMENT_3D('',#179266,#114105,#114106);
#99753=AXIS2_PLACEMENT_3D('',#179270,#114108,#114109);
#99754=AXIS2_PLACEMENT_3D('',#179272,#114110,#114111);
#99755=AXIS2_PLACEMENT_3D('',#179274,#114112,#114113);
#99756=AXIS2_PLACEMENT_3D('',#179276,#114115,#114116);
#99757=AXIS2_PLACEMENT_3D('',#179280,#114118,#114119);
#99758=AXIS2_PLACEMENT_3D('',#179282,#114121,#114122);
#99759=AXIS2_PLACEMENT_3D('',#179283,#114123,#114124);
#99760=AXIS2_PLACEMENT_3D('',#179284,#114125,#114126);
#99761=AXIS2_PLACEMENT_3D('',#179285,#114127,#114128);
#99762=AXIS2_PLACEMENT_3D('',#179286,#114129,#114130);
#99763=AXIS2_PLACEMENT_3D('',#179287,#114131,#114132);
#99764=AXIS2_PLACEMENT_3D('',#179288,#114133,#114134);
#99765=AXIS2_PLACEMENT_3D('',#179289,#114135,#114136);
#99766=AXIS2_PLACEMENT_3D('',#179290,#114137,#114138);
#99767=AXIS2_PLACEMENT_3D('',#179291,#114139,#114140);
#99768=AXIS2_PLACEMENT_3D('',#179292,#114141,#114142);
#99769=AXIS2_PLACEMENT_3D('',#179293,#114143,#114144);
#99770=AXIS2_PLACEMENT_3D('',#179294,#114145,#114146);
#99771=AXIS2_PLACEMENT_3D('',#179297,#114147,#114148);
#99772=AXIS2_PLACEMENT_3D('',#179301,#114150,#114151);
#99773=AXIS2_PLACEMENT_3D('',#179303,#114152,#114153);
#99774=AXIS2_PLACEMENT_3D('',#179305,#114154,#114155);
#99775=AXIS2_PLACEMENT_3D('',#179307,#114157,#114158);
#99776=AXIS2_PLACEMENT_3D('',#179311,#114160,#114161);
#99777=AXIS2_PLACEMENT_3D('',#179313,#114163,#114164);
#99778=AXIS2_PLACEMENT_3D('',#179316,#114165,#114166);
#99779=AXIS2_PLACEMENT_3D('',#179320,#114168,#114169);
#99780=AXIS2_PLACEMENT_3D('',#179322,#114171,#114172);
#99781=AXIS2_PLACEMENT_3D('',#179325,#114173,#114174);
#99782=AXIS2_PLACEMENT_3D('',#179329,#114176,#114177);
#99783=AXIS2_PLACEMENT_3D('',#179331,#114178,#114179);
#99784=AXIS2_PLACEMENT_3D('',#179333,#114180,#114181);
#99785=AXIS2_PLACEMENT_3D('',#179335,#114183,#114184);
#99786=AXIS2_PLACEMENT_3D('',#179339,#114186,#114187);
#99787=AXIS2_PLACEMENT_3D('',#179341,#114189,#114190);
#99788=AXIS2_PLACEMENT_3D('',#179342,#114191,#114192);
#99789=AXIS2_PLACEMENT_3D('',#179343,#114193,#114194);
#99790=AXIS2_PLACEMENT_3D('',#179344,#114195,#114196);
#99791=AXIS2_PLACEMENT_3D('',#179345,#114197,#114198);
#99792=AXIS2_PLACEMENT_3D('',#179346,#114199,#114200);
#99793=AXIS2_PLACEMENT_3D('',#179347,#114201,#114202);
#99794=AXIS2_PLACEMENT_3D('',#179348,#114203,#114204);
#99795=AXIS2_PLACEMENT_3D('',#179349,#114205,#114206);
#99796=AXIS2_PLACEMENT_3D('',#179350,#114207,#114208);
#99797=AXIS2_PLACEMENT_3D('',#179351,#114209,#114210);
#99798=AXIS2_PLACEMENT_3D('',#179352,#114211,#114212);
#99799=AXIS2_PLACEMENT_3D('',#179353,#114213,#114214);
#99800=AXIS2_PLACEMENT_3D('',#179356,#114215,#114216);
#99801=AXIS2_PLACEMENT_3D('',#179360,#114218,#114219);
#99802=AXIS2_PLACEMENT_3D('',#179362,#114220,#114221);
#99803=AXIS2_PLACEMENT_3D('',#179364,#114222,#114223);
#99804=AXIS2_PLACEMENT_3D('',#179366,#114225,#114226);
#99805=AXIS2_PLACEMENT_3D('',#179370,#114228,#114229);
#99806=AXIS2_PLACEMENT_3D('',#179372,#114231,#114232);
#99807=AXIS2_PLACEMENT_3D('',#179375,#114233,#114234);
#99808=AXIS2_PLACEMENT_3D('',#179379,#114236,#114237);
#99809=AXIS2_PLACEMENT_3D('',#179381,#114239,#114240);
#99810=AXIS2_PLACEMENT_3D('',#179384,#114241,#114242);
#99811=AXIS2_PLACEMENT_3D('',#179388,#114244,#114245);
#99812=AXIS2_PLACEMENT_3D('',#179390,#114246,#114247);
#99813=AXIS2_PLACEMENT_3D('',#179392,#114248,#114249);
#99814=AXIS2_PLACEMENT_3D('',#179394,#114251,#114252);
#99815=AXIS2_PLACEMENT_3D('',#179398,#114254,#114255);
#99816=AXIS2_PLACEMENT_3D('',#179400,#114257,#114258);
#99817=AXIS2_PLACEMENT_3D('',#179401,#114259,#114260);
#99818=AXIS2_PLACEMENT_3D('',#179402,#114261,#114262);
#99819=AXIS2_PLACEMENT_3D('',#179403,#114263,#114264);
#99820=AXIS2_PLACEMENT_3D('',#179404,#114265,#114266);
#99821=AXIS2_PLACEMENT_3D('',#179405,#114267,#114268);
#99822=AXIS2_PLACEMENT_3D('',#179406,#114269,#114270);
#99823=AXIS2_PLACEMENT_3D('',#179407,#114271,#114272);
#99824=AXIS2_PLACEMENT_3D('',#179408,#114273,#114274);
#99825=AXIS2_PLACEMENT_3D('',#179409,#114275,#114276);
#99826=AXIS2_PLACEMENT_3D('',#179410,#114277,#114278);
#99827=AXIS2_PLACEMENT_3D('',#179411,#114279,#114280);
#99828=AXIS2_PLACEMENT_3D('',#179412,#114281,#114282);
#99829=AXIS2_PLACEMENT_3D('',#179415,#114283,#114284);
#99830=AXIS2_PLACEMENT_3D('',#179419,#114286,#114287);
#99831=AXIS2_PLACEMENT_3D('',#179421,#114288,#114289);
#99832=AXIS2_PLACEMENT_3D('',#179423,#114290,#114291);
#99833=AXIS2_PLACEMENT_3D('',#179425,#114293,#114294);
#99834=AXIS2_PLACEMENT_3D('',#179429,#114296,#114297);
#99835=AXIS2_PLACEMENT_3D('',#179431,#114299,#114300);
#99836=AXIS2_PLACEMENT_3D('',#179434,#114301,#114302);
#99837=AXIS2_PLACEMENT_3D('',#179438,#114304,#114305);
#99838=AXIS2_PLACEMENT_3D('',#179440,#114307,#114308);
#99839=AXIS2_PLACEMENT_3D('',#179443,#114309,#114310);
#99840=AXIS2_PLACEMENT_3D('',#179447,#114312,#114313);
#99841=AXIS2_PLACEMENT_3D('',#179449,#114314,#114315);
#99842=AXIS2_PLACEMENT_3D('',#179451,#114316,#114317);
#99843=AXIS2_PLACEMENT_3D('',#179453,#114319,#114320);
#99844=AXIS2_PLACEMENT_3D('',#179457,#114322,#114323);
#99845=AXIS2_PLACEMENT_3D('',#179459,#114325,#114326);
#99846=AXIS2_PLACEMENT_3D('',#179460,#114327,#114328);
#99847=AXIS2_PLACEMENT_3D('',#179461,#114329,#114330);
#99848=AXIS2_PLACEMENT_3D('',#179462,#114331,#114332);
#99849=AXIS2_PLACEMENT_3D('',#179463,#114333,#114334);
#99850=AXIS2_PLACEMENT_3D('',#179464,#114335,#114336);
#99851=AXIS2_PLACEMENT_3D('',#179465,#114337,#114338);
#99852=AXIS2_PLACEMENT_3D('',#179466,#114339,#114340);
#99853=AXIS2_PLACEMENT_3D('',#179467,#114341,#114342);
#99854=AXIS2_PLACEMENT_3D('',#179468,#114343,#114344);
#99855=AXIS2_PLACEMENT_3D('',#179469,#114345,#114346);
#99856=AXIS2_PLACEMENT_3D('',#179470,#114347,#114348);
#99857=AXIS2_PLACEMENT_3D('',#179471,#114349,#114350);
#99858=AXIS2_PLACEMENT_3D('',#179474,#114351,#114352);
#99859=AXIS2_PLACEMENT_3D('',#179478,#114354,#114355);
#99860=AXIS2_PLACEMENT_3D('',#179480,#114356,#114357);
#99861=AXIS2_PLACEMENT_3D('',#179482,#114358,#114359);
#99862=AXIS2_PLACEMENT_3D('',#179484,#114361,#114362);
#99863=AXIS2_PLACEMENT_3D('',#179488,#114364,#114365);
#99864=AXIS2_PLACEMENT_3D('',#179490,#114367,#114368);
#99865=AXIS2_PLACEMENT_3D('',#179493,#114369,#114370);
#99866=AXIS2_PLACEMENT_3D('',#179497,#114372,#114373);
#99867=AXIS2_PLACEMENT_3D('',#179499,#114375,#114376);
#99868=AXIS2_PLACEMENT_3D('',#179502,#114377,#114378);
#99869=AXIS2_PLACEMENT_3D('',#179506,#114380,#114381);
#99870=AXIS2_PLACEMENT_3D('',#179508,#114382,#114383);
#99871=AXIS2_PLACEMENT_3D('',#179510,#114384,#114385);
#99872=AXIS2_PLACEMENT_3D('',#179512,#114387,#114388);
#99873=AXIS2_PLACEMENT_3D('',#179516,#114390,#114391);
#99874=AXIS2_PLACEMENT_3D('',#179518,#114393,#114394);
#99875=AXIS2_PLACEMENT_3D('',#179519,#114395,#114396);
#99876=AXIS2_PLACEMENT_3D('',#179520,#114397,#114398);
#99877=AXIS2_PLACEMENT_3D('',#179521,#114399,#114400);
#99878=AXIS2_PLACEMENT_3D('',#179522,#114401,#114402);
#99879=AXIS2_PLACEMENT_3D('',#179523,#114403,#114404);
#99880=AXIS2_PLACEMENT_3D('',#179524,#114405,#114406);
#99881=AXIS2_PLACEMENT_3D('',#179525,#114407,#114408);
#99882=AXIS2_PLACEMENT_3D('',#179526,#114409,#114410);
#99883=AXIS2_PLACEMENT_3D('',#179527,#114411,#114412);
#99884=AXIS2_PLACEMENT_3D('',#179528,#114413,#114414);
#99885=AXIS2_PLACEMENT_3D('',#179529,#114415,#114416);
#99886=AXIS2_PLACEMENT_3D('',#179530,#114417,#114418);
#99887=AXIS2_PLACEMENT_3D('',#179533,#114419,#114420);
#99888=AXIS2_PLACEMENT_3D('',#179537,#114422,#114423);
#99889=AXIS2_PLACEMENT_3D('',#179539,#114424,#114425);
#99890=AXIS2_PLACEMENT_3D('',#179541,#114426,#114427);
#99891=AXIS2_PLACEMENT_3D('',#179543,#114429,#114430);
#99892=AXIS2_PLACEMENT_3D('',#179547,#114432,#114433);
#99893=AXIS2_PLACEMENT_3D('',#179549,#114435,#114436);
#99894=AXIS2_PLACEMENT_3D('',#179552,#114437,#114438);
#99895=AXIS2_PLACEMENT_3D('',#179556,#114440,#114441);
#99896=AXIS2_PLACEMENT_3D('',#179558,#114443,#114444);
#99897=AXIS2_PLACEMENT_3D('',#179561,#114445,#114446);
#99898=AXIS2_PLACEMENT_3D('',#179565,#114448,#114449);
#99899=AXIS2_PLACEMENT_3D('',#179567,#114450,#114451);
#99900=AXIS2_PLACEMENT_3D('',#179569,#114452,#114453);
#99901=AXIS2_PLACEMENT_3D('',#179571,#114455,#114456);
#99902=AXIS2_PLACEMENT_3D('',#179575,#114458,#114459);
#99903=AXIS2_PLACEMENT_3D('',#179577,#114461,#114462);
#99904=AXIS2_PLACEMENT_3D('',#179578,#114463,#114464);
#99905=AXIS2_PLACEMENT_3D('',#179579,#114465,#114466);
#99906=AXIS2_PLACEMENT_3D('',#179580,#114467,#114468);
#99907=AXIS2_PLACEMENT_3D('',#179581,#114469,#114470);
#99908=AXIS2_PLACEMENT_3D('',#179582,#114471,#114472);
#99909=AXIS2_PLACEMENT_3D('',#179583,#114473,#114474);
#99910=AXIS2_PLACEMENT_3D('',#179584,#114475,#114476);
#99911=AXIS2_PLACEMENT_3D('',#179585,#114477,#114478);
#99912=AXIS2_PLACEMENT_3D('',#179586,#114479,#114480);
#99913=AXIS2_PLACEMENT_3D('',#179587,#114481,#114482);
#99914=AXIS2_PLACEMENT_3D('',#179588,#114483,#114484);
#99915=AXIS2_PLACEMENT_3D('',#179589,#114485,#114486);
#99916=AXIS2_PLACEMENT_3D('',#179592,#114487,#114488);
#99917=AXIS2_PLACEMENT_3D('',#179596,#114490,#114491);
#99918=AXIS2_PLACEMENT_3D('',#179598,#114492,#114493);
#99919=AXIS2_PLACEMENT_3D('',#179600,#114494,#114495);
#99920=AXIS2_PLACEMENT_3D('',#179602,#114497,#114498);
#99921=AXIS2_PLACEMENT_3D('',#179606,#114500,#114501);
#99922=AXIS2_PLACEMENT_3D('',#179608,#114503,#114504);
#99923=AXIS2_PLACEMENT_3D('',#179611,#114505,#114506);
#99924=AXIS2_PLACEMENT_3D('',#179615,#114508,#114509);
#99925=AXIS2_PLACEMENT_3D('',#179617,#114511,#114512);
#99926=AXIS2_PLACEMENT_3D('',#179620,#114513,#114514);
#99927=AXIS2_PLACEMENT_3D('',#179624,#114516,#114517);
#99928=AXIS2_PLACEMENT_3D('',#179626,#114518,#114519);
#99929=AXIS2_PLACEMENT_3D('',#179628,#114520,#114521);
#99930=AXIS2_PLACEMENT_3D('',#179630,#114523,#114524);
#99931=AXIS2_PLACEMENT_3D('',#179634,#114526,#114527);
#99932=AXIS2_PLACEMENT_3D('',#179636,#114529,#114530);
#99933=AXIS2_PLACEMENT_3D('',#179637,#114531,#114532);
#99934=AXIS2_PLACEMENT_3D('',#179638,#114533,#114534);
#99935=AXIS2_PLACEMENT_3D('',#179639,#114535,#114536);
#99936=AXIS2_PLACEMENT_3D('',#179640,#114537,#114538);
#99937=AXIS2_PLACEMENT_3D('',#179641,#114539,#114540);
#99938=AXIS2_PLACEMENT_3D('',#179642,#114541,#114542);
#99939=AXIS2_PLACEMENT_3D('',#179643,#114543,#114544);
#99940=AXIS2_PLACEMENT_3D('',#179644,#114545,#114546);
#99941=AXIS2_PLACEMENT_3D('',#179645,#114547,#114548);
#99942=AXIS2_PLACEMENT_3D('',#179646,#114549,#114550);
#99943=AXIS2_PLACEMENT_3D('',#179647,#114551,#114552);
#99944=AXIS2_PLACEMENT_3D('',#179648,#114553,#114554);
#99945=AXIS2_PLACEMENT_3D('',#179651,#114555,#114556);
#99946=AXIS2_PLACEMENT_3D('',#179655,#114558,#114559);
#99947=AXIS2_PLACEMENT_3D('',#179657,#114560,#114561);
#99948=AXIS2_PLACEMENT_3D('',#179659,#114562,#114563);
#99949=AXIS2_PLACEMENT_3D('',#179661,#114565,#114566);
#99950=AXIS2_PLACEMENT_3D('',#179665,#114568,#114569);
#99951=AXIS2_PLACEMENT_3D('',#179667,#114571,#114572);
#99952=AXIS2_PLACEMENT_3D('',#179670,#114573,#114574);
#99953=AXIS2_PLACEMENT_3D('',#179674,#114576,#114577);
#99954=AXIS2_PLACEMENT_3D('',#179676,#114579,#114580);
#99955=AXIS2_PLACEMENT_3D('',#179679,#114581,#114582);
#99956=AXIS2_PLACEMENT_3D('',#179683,#114584,#114585);
#99957=AXIS2_PLACEMENT_3D('',#179685,#114586,#114587);
#99958=AXIS2_PLACEMENT_3D('',#179687,#114588,#114589);
#99959=AXIS2_PLACEMENT_3D('',#179689,#114591,#114592);
#99960=AXIS2_PLACEMENT_3D('',#179693,#114594,#114595);
#99961=AXIS2_PLACEMENT_3D('',#179695,#114597,#114598);
#99962=AXIS2_PLACEMENT_3D('',#179696,#114599,#114600);
#99963=AXIS2_PLACEMENT_3D('',#179697,#114601,#114602);
#99964=AXIS2_PLACEMENT_3D('',#179698,#114603,#114604);
#99965=AXIS2_PLACEMENT_3D('',#179699,#114605,#114606);
#99966=AXIS2_PLACEMENT_3D('',#179700,#114607,#114608);
#99967=AXIS2_PLACEMENT_3D('',#179701,#114609,#114610);
#99968=AXIS2_PLACEMENT_3D('',#179702,#114611,#114612);
#99969=AXIS2_PLACEMENT_3D('',#179703,#114613,#114614);
#99970=AXIS2_PLACEMENT_3D('',#179704,#114615,#114616);
#99971=AXIS2_PLACEMENT_3D('',#179705,#114617,#114618);
#99972=AXIS2_PLACEMENT_3D('',#179706,#114619,#114620);
#99973=AXIS2_PLACEMENT_3D('',#179707,#114621,#114622);
#99974=AXIS2_PLACEMENT_3D('',#179710,#114623,#114624);
#99975=AXIS2_PLACEMENT_3D('',#179714,#114626,#114627);
#99976=AXIS2_PLACEMENT_3D('',#179716,#114628,#114629);
#99977=AXIS2_PLACEMENT_3D('',#179718,#114630,#114631);
#99978=AXIS2_PLACEMENT_3D('',#179720,#114633,#114634);
#99979=AXIS2_PLACEMENT_3D('',#179724,#114636,#114637);
#99980=AXIS2_PLACEMENT_3D('',#179726,#114639,#114640);
#99981=AXIS2_PLACEMENT_3D('',#179729,#114641,#114642);
#99982=AXIS2_PLACEMENT_3D('',#179733,#114644,#114645);
#99983=AXIS2_PLACEMENT_3D('',#179735,#114647,#114648);
#99984=AXIS2_PLACEMENT_3D('',#179738,#114649,#114650);
#99985=AXIS2_PLACEMENT_3D('',#179742,#114652,#114653);
#99986=AXIS2_PLACEMENT_3D('',#179744,#114654,#114655);
#99987=AXIS2_PLACEMENT_3D('',#179746,#114656,#114657);
#99988=AXIS2_PLACEMENT_3D('',#179748,#114659,#114660);
#99989=AXIS2_PLACEMENT_3D('',#179752,#114662,#114663);
#99990=AXIS2_PLACEMENT_3D('',#179754,#114665,#114666);
#99991=AXIS2_PLACEMENT_3D('',#179755,#114667,#114668);
#99992=AXIS2_PLACEMENT_3D('',#179756,#114669,#114670);
#99993=AXIS2_PLACEMENT_3D('',#179757,#114671,#114672);
#99994=AXIS2_PLACEMENT_3D('',#179758,#114673,#114674);
#99995=AXIS2_PLACEMENT_3D('',#179759,#114675,#114676);
#99996=AXIS2_PLACEMENT_3D('',#179760,#114677,#114678);
#99997=AXIS2_PLACEMENT_3D('',#179761,#114679,#114680);
#99998=AXIS2_PLACEMENT_3D('',#179762,#114681,#114682);
#99999=AXIS2_PLACEMENT_3D('',#179763,#114683,#114684);
#100000=AXIS2_PLACEMENT_3D('',#179764,#114685,#114686);
#100001=AXIS2_PLACEMENT_3D('',#179765,#114687,#114688);
#100002=AXIS2_PLACEMENT_3D('',#179766,#114689,#114690);
#100003=AXIS2_PLACEMENT_3D('',#179769,#114691,#114692);
#100004=AXIS2_PLACEMENT_3D('',#179773,#114694,#114695);
#100005=AXIS2_PLACEMENT_3D('',#179775,#114696,#114697);
#100006=AXIS2_PLACEMENT_3D('',#179777,#114698,#114699);
#100007=AXIS2_PLACEMENT_3D('',#179779,#114701,#114702);
#100008=AXIS2_PLACEMENT_3D('',#179783,#114704,#114705);
#100009=AXIS2_PLACEMENT_3D('',#179785,#114707,#114708);
#100010=AXIS2_PLACEMENT_3D('',#179788,#114709,#114710);
#100011=AXIS2_PLACEMENT_3D('',#179792,#114712,#114713);
#100012=AXIS2_PLACEMENT_3D('',#179794,#114715,#114716);
#100013=AXIS2_PLACEMENT_3D('',#179797,#114717,#114718);
#100014=AXIS2_PLACEMENT_3D('',#179801,#114720,#114721);
#100015=AXIS2_PLACEMENT_3D('',#179803,#114722,#114723);
#100016=AXIS2_PLACEMENT_3D('',#179805,#114724,#114725);
#100017=AXIS2_PLACEMENT_3D('',#179807,#114727,#114728);
#100018=AXIS2_PLACEMENT_3D('',#179811,#114730,#114731);
#100019=AXIS2_PLACEMENT_3D('',#179813,#114733,#114734);
#100020=AXIS2_PLACEMENT_3D('',#179814,#114735,#114736);
#100021=AXIS2_PLACEMENT_3D('',#179815,#114737,#114738);
#100022=AXIS2_PLACEMENT_3D('',#179816,#114739,#114740);
#100023=AXIS2_PLACEMENT_3D('',#179817,#114741,#114742);
#100024=AXIS2_PLACEMENT_3D('',#179818,#114743,#114744);
#100025=AXIS2_PLACEMENT_3D('',#179819,#114745,#114746);
#100026=AXIS2_PLACEMENT_3D('',#179820,#114747,#114748);
#100027=AXIS2_PLACEMENT_3D('',#179821,#114749,#114750);
#100028=AXIS2_PLACEMENT_3D('',#179822,#114751,#114752);
#100029=AXIS2_PLACEMENT_3D('',#179823,#114753,#114754);
#100030=AXIS2_PLACEMENT_3D('',#179824,#114755,#114756);
#100031=AXIS2_PLACEMENT_3D('',#179825,#114757,#114758);
#100032=AXIS2_PLACEMENT_3D('',#179828,#114759,#114760);
#100033=AXIS2_PLACEMENT_3D('',#179832,#114762,#114763);
#100034=AXIS2_PLACEMENT_3D('',#179834,#114764,#114765);
#100035=AXIS2_PLACEMENT_3D('',#179836,#114766,#114767);
#100036=AXIS2_PLACEMENT_3D('',#179838,#114769,#114770);
#100037=AXIS2_PLACEMENT_3D('',#179842,#114772,#114773);
#100038=AXIS2_PLACEMENT_3D('',#179844,#114775,#114776);
#100039=AXIS2_PLACEMENT_3D('',#179847,#114777,#114778);
#100040=AXIS2_PLACEMENT_3D('',#179851,#114780,#114781);
#100041=AXIS2_PLACEMENT_3D('',#179853,#114783,#114784);
#100042=AXIS2_PLACEMENT_3D('',#179856,#114785,#114786);
#100043=AXIS2_PLACEMENT_3D('',#179860,#114788,#114789);
#100044=AXIS2_PLACEMENT_3D('',#179862,#114790,#114791);
#100045=AXIS2_PLACEMENT_3D('',#179864,#114792,#114793);
#100046=AXIS2_PLACEMENT_3D('',#179866,#114795,#114796);
#100047=AXIS2_PLACEMENT_3D('',#179870,#114798,#114799);
#100048=AXIS2_PLACEMENT_3D('',#179872,#114801,#114802);
#100049=AXIS2_PLACEMENT_3D('',#179873,#114803,#114804);
#100050=AXIS2_PLACEMENT_3D('',#179874,#114805,#114806);
#100051=AXIS2_PLACEMENT_3D('',#179875,#114807,#114808);
#100052=AXIS2_PLACEMENT_3D('',#179876,#114809,#114810);
#100053=AXIS2_PLACEMENT_3D('',#179877,#114811,#114812);
#100054=AXIS2_PLACEMENT_3D('',#179878,#114813,#114814);
#100055=AXIS2_PLACEMENT_3D('',#179879,#114815,#114816);
#100056=AXIS2_PLACEMENT_3D('',#179880,#114817,#114818);
#100057=AXIS2_PLACEMENT_3D('',#179881,#114819,#114820);
#100058=AXIS2_PLACEMENT_3D('',#179882,#114821,#114822);
#100059=AXIS2_PLACEMENT_3D('',#179883,#114823,#114824);
#100060=AXIS2_PLACEMENT_3D('',#179884,#114825,#114826);
#100061=AXIS2_PLACEMENT_3D('',#179887,#114827,#114828);
#100062=AXIS2_PLACEMENT_3D('',#179891,#114830,#114831);
#100063=AXIS2_PLACEMENT_3D('',#179893,#114832,#114833);
#100064=AXIS2_PLACEMENT_3D('',#179895,#114834,#114835);
#100065=AXIS2_PLACEMENT_3D('',#179897,#114837,#114838);
#100066=AXIS2_PLACEMENT_3D('',#179901,#114840,#114841);
#100067=AXIS2_PLACEMENT_3D('',#179903,#114843,#114844);
#100068=AXIS2_PLACEMENT_3D('',#179906,#114845,#114846);
#100069=AXIS2_PLACEMENT_3D('',#179910,#114848,#114849);
#100070=AXIS2_PLACEMENT_3D('',#179912,#114851,#114852);
#100071=AXIS2_PLACEMENT_3D('',#179915,#114853,#114854);
#100072=AXIS2_PLACEMENT_3D('',#179919,#114856,#114857);
#100073=AXIS2_PLACEMENT_3D('',#179921,#114858,#114859);
#100074=AXIS2_PLACEMENT_3D('',#179923,#114860,#114861);
#100075=AXIS2_PLACEMENT_3D('',#179925,#114863,#114864);
#100076=AXIS2_PLACEMENT_3D('',#179929,#114866,#114867);
#100077=AXIS2_PLACEMENT_3D('',#179931,#114869,#114870);
#100078=AXIS2_PLACEMENT_3D('',#179932,#114871,#114872);
#100079=AXIS2_PLACEMENT_3D('',#179933,#114873,#114874);
#100080=AXIS2_PLACEMENT_3D('',#179934,#114875,#114876);
#100081=AXIS2_PLACEMENT_3D('',#179935,#114877,#114878);
#100082=AXIS2_PLACEMENT_3D('',#179936,#114879,#114880);
#100083=AXIS2_PLACEMENT_3D('',#179937,#114881,#114882);
#100084=AXIS2_PLACEMENT_3D('',#179938,#114883,#114884);
#100085=AXIS2_PLACEMENT_3D('',#179939,#114885,#114886);
#100086=AXIS2_PLACEMENT_3D('',#179940,#114887,#114888);
#100087=AXIS2_PLACEMENT_3D('',#179941,#114889,#114890);
#100088=AXIS2_PLACEMENT_3D('',#179942,#114891,#114892);
#100089=AXIS2_PLACEMENT_3D('',#179943,#114893,#114894);
#100090=AXIS2_PLACEMENT_3D('',#179946,#114895,#114896);
#100091=AXIS2_PLACEMENT_3D('',#179950,#114898,#114899);
#100092=AXIS2_PLACEMENT_3D('',#179952,#114900,#114901);
#100093=AXIS2_PLACEMENT_3D('',#179954,#114902,#114903);
#100094=AXIS2_PLACEMENT_3D('',#179956,#114905,#114906);
#100095=AXIS2_PLACEMENT_3D('',#179960,#114908,#114909);
#100096=AXIS2_PLACEMENT_3D('',#179962,#114911,#114912);
#100097=AXIS2_PLACEMENT_3D('',#179965,#114913,#114914);
#100098=AXIS2_PLACEMENT_3D('',#179969,#114916,#114917);
#100099=AXIS2_PLACEMENT_3D('',#179971,#114919,#114920);
#100100=AXIS2_PLACEMENT_3D('',#179974,#114921,#114922);
#100101=AXIS2_PLACEMENT_3D('',#179978,#114924,#114925);
#100102=AXIS2_PLACEMENT_3D('',#179980,#114926,#114927);
#100103=AXIS2_PLACEMENT_3D('',#179982,#114928,#114929);
#100104=AXIS2_PLACEMENT_3D('',#179984,#114931,#114932);
#100105=AXIS2_PLACEMENT_3D('',#179988,#114934,#114935);
#100106=AXIS2_PLACEMENT_3D('',#179990,#114937,#114938);
#100107=AXIS2_PLACEMENT_3D('',#179991,#114939,#114940);
#100108=AXIS2_PLACEMENT_3D('',#179992,#114941,#114942);
#100109=AXIS2_PLACEMENT_3D('',#179993,#114943,#114944);
#100110=AXIS2_PLACEMENT_3D('',#179994,#114945,#114946);
#100111=AXIS2_PLACEMENT_3D('',#179995,#114947,#114948);
#100112=AXIS2_PLACEMENT_3D('',#179996,#114949,#114950);
#100113=AXIS2_PLACEMENT_3D('',#179997,#114951,#114952);
#100114=AXIS2_PLACEMENT_3D('',#179998,#114953,#114954);
#100115=AXIS2_PLACEMENT_3D('',#179999,#114955,#114956);
#100116=AXIS2_PLACEMENT_3D('',#180000,#114957,#114958);
#100117=AXIS2_PLACEMENT_3D('',#180001,#114959,#114960);
#100118=AXIS2_PLACEMENT_3D('',#180002,#114961,#114962);
#100119=AXIS2_PLACEMENT_3D('',#180005,#114963,#114964);
#100120=AXIS2_PLACEMENT_3D('',#180009,#114966,#114967);
#100121=AXIS2_PLACEMENT_3D('',#180011,#114968,#114969);
#100122=AXIS2_PLACEMENT_3D('',#180013,#114970,#114971);
#100123=AXIS2_PLACEMENT_3D('',#180015,#114973,#114974);
#100124=AXIS2_PLACEMENT_3D('',#180019,#114976,#114977);
#100125=AXIS2_PLACEMENT_3D('',#180021,#114979,#114980);
#100126=AXIS2_PLACEMENT_3D('',#180024,#114981,#114982);
#100127=AXIS2_PLACEMENT_3D('',#180028,#114984,#114985);
#100128=AXIS2_PLACEMENT_3D('',#180030,#114987,#114988);
#100129=AXIS2_PLACEMENT_3D('',#180033,#114989,#114990);
#100130=AXIS2_PLACEMENT_3D('',#180037,#114992,#114993);
#100131=AXIS2_PLACEMENT_3D('',#180039,#114994,#114995);
#100132=AXIS2_PLACEMENT_3D('',#180041,#114996,#114997);
#100133=AXIS2_PLACEMENT_3D('',#180043,#114999,#115000);
#100134=AXIS2_PLACEMENT_3D('',#180047,#115002,#115003);
#100135=AXIS2_PLACEMENT_3D('',#180049,#115005,#115006);
#100136=AXIS2_PLACEMENT_3D('',#180050,#115007,#115008);
#100137=AXIS2_PLACEMENT_3D('',#180051,#115009,#115010);
#100138=AXIS2_PLACEMENT_3D('',#180052,#115011,#115012);
#100139=AXIS2_PLACEMENT_3D('',#180053,#115013,#115014);
#100140=AXIS2_PLACEMENT_3D('',#180054,#115015,#115016);
#100141=AXIS2_PLACEMENT_3D('',#180055,#115017,#115018);
#100142=AXIS2_PLACEMENT_3D('',#180056,#115019,#115020);
#100143=AXIS2_PLACEMENT_3D('',#180057,#115021,#115022);
#100144=AXIS2_PLACEMENT_3D('',#180058,#115023,#115024);
#100145=AXIS2_PLACEMENT_3D('',#180059,#115025,#115026);
#100146=AXIS2_PLACEMENT_3D('',#180060,#115027,#115028);
#100147=AXIS2_PLACEMENT_3D('',#180061,#115029,#115030);
#100148=AXIS2_PLACEMENT_3D('',#180064,#115031,#115032);
#100149=AXIS2_PLACEMENT_3D('',#180068,#115034,#115035);
#100150=AXIS2_PLACEMENT_3D('',#180070,#115036,#115037);
#100151=AXIS2_PLACEMENT_3D('',#180072,#115038,#115039);
#100152=AXIS2_PLACEMENT_3D('',#180074,#115041,#115042);
#100153=AXIS2_PLACEMENT_3D('',#180078,#115044,#115045);
#100154=AXIS2_PLACEMENT_3D('',#180080,#115047,#115048);
#100155=AXIS2_PLACEMENT_3D('',#180083,#115049,#115050);
#100156=AXIS2_PLACEMENT_3D('',#180087,#115052,#115053);
#100157=AXIS2_PLACEMENT_3D('',#180089,#115055,#115056);
#100158=AXIS2_PLACEMENT_3D('',#180092,#115057,#115058);
#100159=AXIS2_PLACEMENT_3D('',#180096,#115060,#115061);
#100160=AXIS2_PLACEMENT_3D('',#180098,#115062,#115063);
#100161=AXIS2_PLACEMENT_3D('',#180100,#115064,#115065);
#100162=AXIS2_PLACEMENT_3D('',#180102,#115067,#115068);
#100163=AXIS2_PLACEMENT_3D('',#180106,#115070,#115071);
#100164=AXIS2_PLACEMENT_3D('',#180108,#115073,#115074);
#100165=AXIS2_PLACEMENT_3D('',#180109,#115075,#115076);
#100166=AXIS2_PLACEMENT_3D('',#180110,#115077,#115078);
#100167=AXIS2_PLACEMENT_3D('',#180111,#115079,#115080);
#100168=AXIS2_PLACEMENT_3D('',#180112,#115081,#115082);
#100169=AXIS2_PLACEMENT_3D('',#180113,#115083,#115084);
#100170=AXIS2_PLACEMENT_3D('',#180114,#115085,#115086);
#100171=AXIS2_PLACEMENT_3D('',#180115,#115087,#115088);
#100172=AXIS2_PLACEMENT_3D('',#180116,#115089,#115090);
#100173=AXIS2_PLACEMENT_3D('',#180117,#115091,#115092);
#100174=AXIS2_PLACEMENT_3D('',#180118,#115093,#115094);
#100175=AXIS2_PLACEMENT_3D('',#180119,#115095,#115096);
#100176=AXIS2_PLACEMENT_3D('',#180120,#115097,#115098);
#100177=AXIS2_PLACEMENT_3D('',#180123,#115099,#115100);
#100178=AXIS2_PLACEMENT_3D('',#180127,#115102,#115103);
#100179=AXIS2_PLACEMENT_3D('',#180129,#115104,#115105);
#100180=AXIS2_PLACEMENT_3D('',#180131,#115106,#115107);
#100181=AXIS2_PLACEMENT_3D('',#180133,#115109,#115110);
#100182=AXIS2_PLACEMENT_3D('',#180137,#115112,#115113);
#100183=AXIS2_PLACEMENT_3D('',#180139,#115115,#115116);
#100184=AXIS2_PLACEMENT_3D('',#180142,#115117,#115118);
#100185=AXIS2_PLACEMENT_3D('',#180146,#115120,#115121);
#100186=AXIS2_PLACEMENT_3D('',#180148,#115123,#115124);
#100187=AXIS2_PLACEMENT_3D('',#180151,#115125,#115126);
#100188=AXIS2_PLACEMENT_3D('',#180155,#115128,#115129);
#100189=AXIS2_PLACEMENT_3D('',#180157,#115130,#115131);
#100190=AXIS2_PLACEMENT_3D('',#180159,#115132,#115133);
#100191=AXIS2_PLACEMENT_3D('',#180161,#115135,#115136);
#100192=AXIS2_PLACEMENT_3D('',#180165,#115138,#115139);
#100193=AXIS2_PLACEMENT_3D('',#180167,#115141,#115142);
#100194=AXIS2_PLACEMENT_3D('',#180168,#115143,#115144);
#100195=AXIS2_PLACEMENT_3D('',#180169,#115145,#115146);
#100196=AXIS2_PLACEMENT_3D('',#180170,#115147,#115148);
#100197=AXIS2_PLACEMENT_3D('',#180171,#115149,#115150);
#100198=AXIS2_PLACEMENT_3D('',#180172,#115151,#115152);
#100199=AXIS2_PLACEMENT_3D('',#180173,#115153,#115154);
#100200=AXIS2_PLACEMENT_3D('',#180174,#115155,#115156);
#100201=AXIS2_PLACEMENT_3D('',#180175,#115157,#115158);
#100202=AXIS2_PLACEMENT_3D('',#180176,#115159,#115160);
#100203=AXIS2_PLACEMENT_3D('',#180177,#115161,#115162);
#100204=AXIS2_PLACEMENT_3D('',#180178,#115163,#115164);
#100205=AXIS2_PLACEMENT_3D('',#180179,#115165,#115166);
#100206=AXIS2_PLACEMENT_3D('',#180182,#115167,#115168);
#100207=AXIS2_PLACEMENT_3D('',#180186,#115170,#115171);
#100208=AXIS2_PLACEMENT_3D('',#180188,#115172,#115173);
#100209=AXIS2_PLACEMENT_3D('',#180190,#115174,#115175);
#100210=AXIS2_PLACEMENT_3D('',#180192,#115177,#115178);
#100211=AXIS2_PLACEMENT_3D('',#180196,#115180,#115181);
#100212=AXIS2_PLACEMENT_3D('',#180198,#115183,#115184);
#100213=AXIS2_PLACEMENT_3D('',#180201,#115185,#115186);
#100214=AXIS2_PLACEMENT_3D('',#180205,#115188,#115189);
#100215=AXIS2_PLACEMENT_3D('',#180207,#115191,#115192);
#100216=AXIS2_PLACEMENT_3D('',#180210,#115193,#115194);
#100217=AXIS2_PLACEMENT_3D('',#180214,#115196,#115197);
#100218=AXIS2_PLACEMENT_3D('',#180216,#115198,#115199);
#100219=AXIS2_PLACEMENT_3D('',#180218,#115200,#115201);
#100220=AXIS2_PLACEMENT_3D('',#180220,#115203,#115204);
#100221=AXIS2_PLACEMENT_3D('',#180224,#115206,#115207);
#100222=AXIS2_PLACEMENT_3D('',#180226,#115209,#115210);
#100223=AXIS2_PLACEMENT_3D('',#180227,#115211,#115212);
#100224=AXIS2_PLACEMENT_3D('',#180228,#115213,#115214);
#100225=AXIS2_PLACEMENT_3D('',#180229,#115215,#115216);
#100226=AXIS2_PLACEMENT_3D('',#180230,#115217,#115218);
#100227=AXIS2_PLACEMENT_3D('',#180231,#115219,#115220);
#100228=AXIS2_PLACEMENT_3D('',#180232,#115221,#115222);
#100229=AXIS2_PLACEMENT_3D('',#180233,#115223,#115224);
#100230=AXIS2_PLACEMENT_3D('',#180234,#115225,#115226);
#100231=AXIS2_PLACEMENT_3D('',#180235,#115227,#115228);
#100232=AXIS2_PLACEMENT_3D('',#180236,#115229,#115230);
#100233=AXIS2_PLACEMENT_3D('',#180237,#115231,#115232);
#100234=AXIS2_PLACEMENT_3D('',#180238,#115233,#115234);
#100235=AXIS2_PLACEMENT_3D('',#180241,#115235,#115236);
#100236=AXIS2_PLACEMENT_3D('',#180245,#115238,#115239);
#100237=AXIS2_PLACEMENT_3D('',#180247,#115240,#115241);
#100238=AXIS2_PLACEMENT_3D('',#180249,#115242,#115243);
#100239=AXIS2_PLACEMENT_3D('',#180251,#115245,#115246);
#100240=AXIS2_PLACEMENT_3D('',#180255,#115248,#115249);
#100241=AXIS2_PLACEMENT_3D('',#180257,#115251,#115252);
#100242=AXIS2_PLACEMENT_3D('',#180260,#115253,#115254);
#100243=AXIS2_PLACEMENT_3D('',#180264,#115256,#115257);
#100244=AXIS2_PLACEMENT_3D('',#180266,#115259,#115260);
#100245=AXIS2_PLACEMENT_3D('',#180269,#115261,#115262);
#100246=AXIS2_PLACEMENT_3D('',#180273,#115264,#115265);
#100247=AXIS2_PLACEMENT_3D('',#180275,#115266,#115267);
#100248=AXIS2_PLACEMENT_3D('',#180277,#115268,#115269);
#100249=AXIS2_PLACEMENT_3D('',#180279,#115271,#115272);
#100250=AXIS2_PLACEMENT_3D('',#180283,#115274,#115275);
#100251=AXIS2_PLACEMENT_3D('',#180285,#115277,#115278);
#100252=AXIS2_PLACEMENT_3D('',#180286,#115279,#115280);
#100253=AXIS2_PLACEMENT_3D('',#180287,#115281,#115282);
#100254=AXIS2_PLACEMENT_3D('',#180288,#115283,#115284);
#100255=AXIS2_PLACEMENT_3D('',#180289,#115285,#115286);
#100256=AXIS2_PLACEMENT_3D('',#180290,#115287,#115288);
#100257=AXIS2_PLACEMENT_3D('',#180291,#115289,#115290);
#100258=AXIS2_PLACEMENT_3D('',#180292,#115291,#115292);
#100259=AXIS2_PLACEMENT_3D('',#180293,#115293,#115294);
#100260=AXIS2_PLACEMENT_3D('',#180294,#115295,#115296);
#100261=AXIS2_PLACEMENT_3D('',#180295,#115297,#115298);
#100262=AXIS2_PLACEMENT_3D('',#180296,#115299,#115300);
#100263=AXIS2_PLACEMENT_3D('',#180297,#115301,#115302);
#100264=AXIS2_PLACEMENT_3D('',#180300,#115303,#115304);
#100265=AXIS2_PLACEMENT_3D('',#180304,#115306,#115307);
#100266=AXIS2_PLACEMENT_3D('',#180306,#115308,#115309);
#100267=AXIS2_PLACEMENT_3D('',#180308,#115310,#115311);
#100268=AXIS2_PLACEMENT_3D('',#180310,#115313,#115314);
#100269=AXIS2_PLACEMENT_3D('',#180314,#115316,#115317);
#100270=AXIS2_PLACEMENT_3D('',#180316,#115319,#115320);
#100271=AXIS2_PLACEMENT_3D('',#180319,#115321,#115322);
#100272=AXIS2_PLACEMENT_3D('',#180323,#115324,#115325);
#100273=AXIS2_PLACEMENT_3D('',#180325,#115327,#115328);
#100274=AXIS2_PLACEMENT_3D('',#180328,#115329,#115330);
#100275=AXIS2_PLACEMENT_3D('',#180332,#115332,#115333);
#100276=AXIS2_PLACEMENT_3D('',#180334,#115334,#115335);
#100277=AXIS2_PLACEMENT_3D('',#180336,#115336,#115337);
#100278=AXIS2_PLACEMENT_3D('',#180338,#115339,#115340);
#100279=AXIS2_PLACEMENT_3D('',#180342,#115342,#115343);
#100280=AXIS2_PLACEMENT_3D('',#180344,#115345,#115346);
#100281=AXIS2_PLACEMENT_3D('',#180345,#115347,#115348);
#100282=AXIS2_PLACEMENT_3D('',#180346,#115349,#115350);
#100283=AXIS2_PLACEMENT_3D('',#180347,#115351,#115352);
#100284=AXIS2_PLACEMENT_3D('',#180348,#115353,#115354);
#100285=AXIS2_PLACEMENT_3D('',#180349,#115355,#115356);
#100286=AXIS2_PLACEMENT_3D('',#180350,#115357,#115358);
#100287=AXIS2_PLACEMENT_3D('',#180351,#115359,#115360);
#100288=AXIS2_PLACEMENT_3D('',#180352,#115361,#115362);
#100289=AXIS2_PLACEMENT_3D('',#180353,#115363,#115364);
#100290=AXIS2_PLACEMENT_3D('',#180354,#115365,#115366);
#100291=AXIS2_PLACEMENT_3D('',#180355,#115367,#115368);
#100292=AXIS2_PLACEMENT_3D('',#180356,#115369,#115370);
#100293=AXIS2_PLACEMENT_3D('',#180359,#115371,#115372);
#100294=AXIS2_PLACEMENT_3D('',#180363,#115374,#115375);
#100295=AXIS2_PLACEMENT_3D('',#180365,#115376,#115377);
#100296=AXIS2_PLACEMENT_3D('',#180367,#115378,#115379);
#100297=AXIS2_PLACEMENT_3D('',#180369,#115381,#115382);
#100298=AXIS2_PLACEMENT_3D('',#180373,#115384,#115385);
#100299=AXIS2_PLACEMENT_3D('',#180375,#115387,#115388);
#100300=AXIS2_PLACEMENT_3D('',#180378,#115389,#115390);
#100301=AXIS2_PLACEMENT_3D('',#180382,#115392,#115393);
#100302=AXIS2_PLACEMENT_3D('',#180384,#115395,#115396);
#100303=AXIS2_PLACEMENT_3D('',#180387,#115397,#115398);
#100304=AXIS2_PLACEMENT_3D('',#180391,#115400,#115401);
#100305=AXIS2_PLACEMENT_3D('',#180393,#115402,#115403);
#100306=AXIS2_PLACEMENT_3D('',#180395,#115404,#115405);
#100307=AXIS2_PLACEMENT_3D('',#180397,#115407,#115408);
#100308=AXIS2_PLACEMENT_3D('',#180401,#115410,#115411);
#100309=AXIS2_PLACEMENT_3D('',#180403,#115413,#115414);
#100310=AXIS2_PLACEMENT_3D('',#180404,#115415,#115416);
#100311=AXIS2_PLACEMENT_3D('',#180405,#115417,#115418);
#100312=AXIS2_PLACEMENT_3D('',#180406,#115419,#115420);
#100313=AXIS2_PLACEMENT_3D('',#180407,#115421,#115422);
#100314=AXIS2_PLACEMENT_3D('',#180408,#115423,#115424);
#100315=AXIS2_PLACEMENT_3D('',#180409,#115425,#115426);
#100316=AXIS2_PLACEMENT_3D('',#180410,#115427,#115428);
#100317=AXIS2_PLACEMENT_3D('',#180411,#115429,#115430);
#100318=AXIS2_PLACEMENT_3D('',#180412,#115431,#115432);
#100319=AXIS2_PLACEMENT_3D('',#180413,#115433,#115434);
#100320=AXIS2_PLACEMENT_3D('',#180414,#115435,#115436);
#100321=AXIS2_PLACEMENT_3D('',#180415,#115437,#115438);
#100322=AXIS2_PLACEMENT_3D('',#180418,#115439,#115440);
#100323=AXIS2_PLACEMENT_3D('',#180422,#115442,#115443);
#100324=AXIS2_PLACEMENT_3D('',#180424,#115444,#115445);
#100325=AXIS2_PLACEMENT_3D('',#180426,#115446,#115447);
#100326=AXIS2_PLACEMENT_3D('',#180428,#115449,#115450);
#100327=AXIS2_PLACEMENT_3D('',#180432,#115452,#115453);
#100328=AXIS2_PLACEMENT_3D('',#180434,#115455,#115456);
#100329=AXIS2_PLACEMENT_3D('',#180437,#115457,#115458);
#100330=AXIS2_PLACEMENT_3D('',#180441,#115460,#115461);
#100331=AXIS2_PLACEMENT_3D('',#180443,#115463,#115464);
#100332=AXIS2_PLACEMENT_3D('',#180446,#115465,#115466);
#100333=AXIS2_PLACEMENT_3D('',#180450,#115468,#115469);
#100334=AXIS2_PLACEMENT_3D('',#180452,#115470,#115471);
#100335=AXIS2_PLACEMENT_3D('',#180454,#115472,#115473);
#100336=AXIS2_PLACEMENT_3D('',#180456,#115475,#115476);
#100337=AXIS2_PLACEMENT_3D('',#180460,#115478,#115479);
#100338=AXIS2_PLACEMENT_3D('',#180462,#115481,#115482);
#100339=AXIS2_PLACEMENT_3D('',#180463,#115483,#115484);
#100340=AXIS2_PLACEMENT_3D('',#180464,#115485,#115486);
#100341=AXIS2_PLACEMENT_3D('',#180465,#115487,#115488);
#100342=AXIS2_PLACEMENT_3D('',#180466,#115489,#115490);
#100343=AXIS2_PLACEMENT_3D('',#180467,#115491,#115492);
#100344=AXIS2_PLACEMENT_3D('',#180468,#115493,#115494);
#100345=AXIS2_PLACEMENT_3D('',#180469,#115495,#115496);
#100346=AXIS2_PLACEMENT_3D('',#180470,#115497,#115498);
#100347=AXIS2_PLACEMENT_3D('',#180471,#115499,#115500);
#100348=AXIS2_PLACEMENT_3D('',#180472,#115501,#115502);
#100349=AXIS2_PLACEMENT_3D('',#180473,#115503,#115504);
#100350=AXIS2_PLACEMENT_3D('',#180474,#115505,#115506);
#100351=AXIS2_PLACEMENT_3D('',#180477,#115507,#115508);
#100352=AXIS2_PLACEMENT_3D('',#180481,#115510,#115511);
#100353=AXIS2_PLACEMENT_3D('',#180483,#115512,#115513);
#100354=AXIS2_PLACEMENT_3D('',#180485,#115514,#115515);
#100355=AXIS2_PLACEMENT_3D('',#180487,#115517,#115518);
#100356=AXIS2_PLACEMENT_3D('',#180491,#115520,#115521);
#100357=AXIS2_PLACEMENT_3D('',#180493,#115523,#115524);
#100358=AXIS2_PLACEMENT_3D('',#180496,#115525,#115526);
#100359=AXIS2_PLACEMENT_3D('',#180500,#115528,#115529);
#100360=AXIS2_PLACEMENT_3D('',#180502,#115531,#115532);
#100361=AXIS2_PLACEMENT_3D('',#180505,#115533,#115534);
#100362=AXIS2_PLACEMENT_3D('',#180509,#115536,#115537);
#100363=AXIS2_PLACEMENT_3D('',#180511,#115538,#115539);
#100364=AXIS2_PLACEMENT_3D('',#180513,#115540,#115541);
#100365=AXIS2_PLACEMENT_3D('',#180515,#115543,#115544);
#100366=AXIS2_PLACEMENT_3D('',#180519,#115546,#115547);
#100367=AXIS2_PLACEMENT_3D('',#180521,#115549,#115550);
#100368=AXIS2_PLACEMENT_3D('',#180522,#115551,#115552);
#100369=AXIS2_PLACEMENT_3D('',#180523,#115553,#115554);
#100370=AXIS2_PLACEMENT_3D('',#180524,#115555,#115556);
#100371=AXIS2_PLACEMENT_3D('',#180525,#115557,#115558);
#100372=AXIS2_PLACEMENT_3D('',#180526,#115559,#115560);
#100373=AXIS2_PLACEMENT_3D('',#180527,#115561,#115562);
#100374=AXIS2_PLACEMENT_3D('',#180528,#115563,#115564);
#100375=AXIS2_PLACEMENT_3D('',#180529,#115565,#115566);
#100376=AXIS2_PLACEMENT_3D('',#180530,#115567,#115568);
#100377=AXIS2_PLACEMENT_3D('',#180531,#115569,#115570);
#100378=AXIS2_PLACEMENT_3D('',#180532,#115571,#115572);
#100379=AXIS2_PLACEMENT_3D('',#180533,#115573,#115574);
#100380=AXIS2_PLACEMENT_3D('',#180536,#115575,#115576);
#100381=AXIS2_PLACEMENT_3D('',#180540,#115578,#115579);
#100382=AXIS2_PLACEMENT_3D('',#180542,#115580,#115581);
#100383=AXIS2_PLACEMENT_3D('',#180544,#115582,#115583);
#100384=AXIS2_PLACEMENT_3D('',#180546,#115585,#115586);
#100385=AXIS2_PLACEMENT_3D('',#180550,#115588,#115589);
#100386=AXIS2_PLACEMENT_3D('',#180552,#115591,#115592);
#100387=AXIS2_PLACEMENT_3D('',#180555,#115593,#115594);
#100388=AXIS2_PLACEMENT_3D('',#180559,#115596,#115597);
#100389=AXIS2_PLACEMENT_3D('',#180561,#115599,#115600);
#100390=AXIS2_PLACEMENT_3D('',#180564,#115601,#115602);
#100391=AXIS2_PLACEMENT_3D('',#180568,#115604,#115605);
#100392=AXIS2_PLACEMENT_3D('',#180570,#115606,#115607);
#100393=AXIS2_PLACEMENT_3D('',#180572,#115608,#115609);
#100394=AXIS2_PLACEMENT_3D('',#180574,#115611,#115612);
#100395=AXIS2_PLACEMENT_3D('',#180578,#115614,#115615);
#100396=AXIS2_PLACEMENT_3D('',#180580,#115617,#115618);
#100397=AXIS2_PLACEMENT_3D('',#180581,#115619,#115620);
#100398=AXIS2_PLACEMENT_3D('',#180582,#115621,#115622);
#100399=AXIS2_PLACEMENT_3D('',#180583,#115623,#115624);
#100400=AXIS2_PLACEMENT_3D('',#180584,#115625,#115626);
#100401=AXIS2_PLACEMENT_3D('',#180585,#115627,#115628);
#100402=AXIS2_PLACEMENT_3D('',#180586,#115629,#115630);
#100403=AXIS2_PLACEMENT_3D('',#180587,#115631,#115632);
#100404=AXIS2_PLACEMENT_3D('',#180588,#115633,#115634);
#100405=AXIS2_PLACEMENT_3D('',#180589,#115635,#115636);
#100406=AXIS2_PLACEMENT_3D('',#180590,#115637,#115638);
#100407=AXIS2_PLACEMENT_3D('',#180591,#115639,#115640);
#100408=AXIS2_PLACEMENT_3D('',#180592,#115641,#115642);
#100409=AXIS2_PLACEMENT_3D('',#180595,#115643,#115644);
#100410=AXIS2_PLACEMENT_3D('',#180599,#115646,#115647);
#100411=AXIS2_PLACEMENT_3D('',#180601,#115648,#115649);
#100412=AXIS2_PLACEMENT_3D('',#180603,#115650,#115651);
#100413=AXIS2_PLACEMENT_3D('',#180605,#115653,#115654);
#100414=AXIS2_PLACEMENT_3D('',#180609,#115656,#115657);
#100415=AXIS2_PLACEMENT_3D('',#180611,#115659,#115660);
#100416=AXIS2_PLACEMENT_3D('',#180614,#115661,#115662);
#100417=AXIS2_PLACEMENT_3D('',#180618,#115664,#115665);
#100418=AXIS2_PLACEMENT_3D('',#180620,#115667,#115668);
#100419=AXIS2_PLACEMENT_3D('',#180623,#115669,#115670);
#100420=AXIS2_PLACEMENT_3D('',#180627,#115672,#115673);
#100421=AXIS2_PLACEMENT_3D('',#180629,#115674,#115675);
#100422=AXIS2_PLACEMENT_3D('',#180631,#115676,#115677);
#100423=AXIS2_PLACEMENT_3D('',#180633,#115679,#115680);
#100424=AXIS2_PLACEMENT_3D('',#180637,#115682,#115683);
#100425=AXIS2_PLACEMENT_3D('',#180639,#115685,#115686);
#100426=AXIS2_PLACEMENT_3D('',#180640,#115687,#115688);
#100427=AXIS2_PLACEMENT_3D('',#180641,#115689,#115690);
#100428=AXIS2_PLACEMENT_3D('',#180642,#115691,#115692);
#100429=AXIS2_PLACEMENT_3D('',#180643,#115693,#115694);
#100430=AXIS2_PLACEMENT_3D('',#180644,#115695,#115696);
#100431=AXIS2_PLACEMENT_3D('',#180645,#115697,#115698);
#100432=AXIS2_PLACEMENT_3D('',#180646,#115699,#115700);
#100433=AXIS2_PLACEMENT_3D('',#180647,#115701,#115702);
#100434=AXIS2_PLACEMENT_3D('',#180648,#115703,#115704);
#100435=AXIS2_PLACEMENT_3D('',#180649,#115705,#115706);
#100436=AXIS2_PLACEMENT_3D('',#180650,#115707,#115708);
#100437=AXIS2_PLACEMENT_3D('',#180651,#115709,#115710);
#100438=AXIS2_PLACEMENT_3D('',#180654,#115711,#115712);
#100439=AXIS2_PLACEMENT_3D('',#180658,#115714,#115715);
#100440=AXIS2_PLACEMENT_3D('',#180660,#115716,#115717);
#100441=AXIS2_PLACEMENT_3D('',#180662,#115718,#115719);
#100442=AXIS2_PLACEMENT_3D('',#180664,#115721,#115722);
#100443=AXIS2_PLACEMENT_3D('',#180668,#115724,#115725);
#100444=AXIS2_PLACEMENT_3D('',#180670,#115727,#115728);
#100445=AXIS2_PLACEMENT_3D('',#180673,#115729,#115730);
#100446=AXIS2_PLACEMENT_3D('',#180677,#115732,#115733);
#100447=AXIS2_PLACEMENT_3D('',#180679,#115735,#115736);
#100448=AXIS2_PLACEMENT_3D('',#180682,#115737,#115738);
#100449=AXIS2_PLACEMENT_3D('',#180686,#115740,#115741);
#100450=AXIS2_PLACEMENT_3D('',#180688,#115742,#115743);
#100451=AXIS2_PLACEMENT_3D('',#180690,#115744,#115745);
#100452=AXIS2_PLACEMENT_3D('',#180692,#115747,#115748);
#100453=AXIS2_PLACEMENT_3D('',#180696,#115750,#115751);
#100454=AXIS2_PLACEMENT_3D('',#180698,#115753,#115754);
#100455=AXIS2_PLACEMENT_3D('',#180699,#115755,#115756);
#100456=AXIS2_PLACEMENT_3D('',#180700,#115757,#115758);
#100457=AXIS2_PLACEMENT_3D('',#180701,#115759,#115760);
#100458=AXIS2_PLACEMENT_3D('',#180702,#115761,#115762);
#100459=AXIS2_PLACEMENT_3D('',#180703,#115763,#115764);
#100460=AXIS2_PLACEMENT_3D('',#180704,#115765,#115766);
#100461=AXIS2_PLACEMENT_3D('',#180705,#115767,#115768);
#100462=AXIS2_PLACEMENT_3D('',#180706,#115769,#115770);
#100463=AXIS2_PLACEMENT_3D('',#180707,#115771,#115772);
#100464=AXIS2_PLACEMENT_3D('',#180708,#115773,#115774);
#100465=AXIS2_PLACEMENT_3D('',#180709,#115775,#115776);
#100466=AXIS2_PLACEMENT_3D('',#180710,#115777,#115778);
#100467=AXIS2_PLACEMENT_3D('',#180713,#115779,#115780);
#100468=AXIS2_PLACEMENT_3D('',#180717,#115782,#115783);
#100469=AXIS2_PLACEMENT_3D('',#180719,#115784,#115785);
#100470=AXIS2_PLACEMENT_3D('',#180721,#115786,#115787);
#100471=AXIS2_PLACEMENT_3D('',#180723,#115789,#115790);
#100472=AXIS2_PLACEMENT_3D('',#180727,#115792,#115793);
#100473=AXIS2_PLACEMENT_3D('',#180729,#115795,#115796);
#100474=AXIS2_PLACEMENT_3D('',#180732,#115797,#115798);
#100475=AXIS2_PLACEMENT_3D('',#180736,#115800,#115801);
#100476=AXIS2_PLACEMENT_3D('',#180738,#115803,#115804);
#100477=AXIS2_PLACEMENT_3D('',#180741,#115805,#115806);
#100478=AXIS2_PLACEMENT_3D('',#180745,#115808,#115809);
#100479=AXIS2_PLACEMENT_3D('',#180747,#115810,#115811);
#100480=AXIS2_PLACEMENT_3D('',#180749,#115812,#115813);
#100481=AXIS2_PLACEMENT_3D('',#180751,#115815,#115816);
#100482=AXIS2_PLACEMENT_3D('',#180755,#115818,#115819);
#100483=AXIS2_PLACEMENT_3D('',#180757,#115821,#115822);
#100484=AXIS2_PLACEMENT_3D('',#180758,#115823,#115824);
#100485=AXIS2_PLACEMENT_3D('',#180759,#115825,#115826);
#100486=AXIS2_PLACEMENT_3D('',#180760,#115827,#115828);
#100487=AXIS2_PLACEMENT_3D('',#180761,#115829,#115830);
#100488=AXIS2_PLACEMENT_3D('',#180762,#115831,#115832);
#100489=AXIS2_PLACEMENT_3D('',#180763,#115833,#115834);
#100490=AXIS2_PLACEMENT_3D('',#180764,#115835,#115836);
#100491=AXIS2_PLACEMENT_3D('',#180765,#115837,#115838);
#100492=AXIS2_PLACEMENT_3D('',#180766,#115839,#115840);
#100493=AXIS2_PLACEMENT_3D('',#180767,#115841,#115842);
#100494=AXIS2_PLACEMENT_3D('',#180768,#115843,#115844);
#100495=AXIS2_PLACEMENT_3D('',#180769,#115845,#115846);
#100496=AXIS2_PLACEMENT_3D('',#180772,#115847,#115848);
#100497=AXIS2_PLACEMENT_3D('',#180776,#115850,#115851);
#100498=AXIS2_PLACEMENT_3D('',#180778,#115852,#115853);
#100499=AXIS2_PLACEMENT_3D('',#180780,#115854,#115855);
#100500=AXIS2_PLACEMENT_3D('',#180782,#115857,#115858);
#100501=AXIS2_PLACEMENT_3D('',#180786,#115860,#115861);
#100502=AXIS2_PLACEMENT_3D('',#180788,#115863,#115864);
#100503=AXIS2_PLACEMENT_3D('',#180791,#115865,#115866);
#100504=AXIS2_PLACEMENT_3D('',#180795,#115868,#115869);
#100505=AXIS2_PLACEMENT_3D('',#180797,#115871,#115872);
#100506=AXIS2_PLACEMENT_3D('',#180800,#115873,#115874);
#100507=AXIS2_PLACEMENT_3D('',#180804,#115876,#115877);
#100508=AXIS2_PLACEMENT_3D('',#180806,#115878,#115879);
#100509=AXIS2_PLACEMENT_3D('',#180808,#115880,#115881);
#100510=AXIS2_PLACEMENT_3D('',#180810,#115883,#115884);
#100511=AXIS2_PLACEMENT_3D('',#180814,#115886,#115887);
#100512=AXIS2_PLACEMENT_3D('',#180816,#115889,#115890);
#100513=AXIS2_PLACEMENT_3D('',#180817,#115891,#115892);
#100514=AXIS2_PLACEMENT_3D('',#180818,#115893,#115894);
#100515=AXIS2_PLACEMENT_3D('',#180819,#115895,#115896);
#100516=AXIS2_PLACEMENT_3D('',#180820,#115897,#115898);
#100517=AXIS2_PLACEMENT_3D('',#180821,#115899,#115900);
#100518=AXIS2_PLACEMENT_3D('',#180822,#115901,#115902);
#100519=AXIS2_PLACEMENT_3D('',#180823,#115903,#115904);
#100520=AXIS2_PLACEMENT_3D('',#180824,#115905,#115906);
#100521=AXIS2_PLACEMENT_3D('',#180825,#115907,#115908);
#100522=AXIS2_PLACEMENT_3D('',#180826,#115909,#115910);
#100523=AXIS2_PLACEMENT_3D('',#180827,#115911,#115912);
#100524=AXIS2_PLACEMENT_3D('',#180828,#115913,#115914);
#100525=AXIS2_PLACEMENT_3D('',#180831,#115915,#115916);
#100526=AXIS2_PLACEMENT_3D('',#180835,#115918,#115919);
#100527=AXIS2_PLACEMENT_3D('',#180837,#115920,#115921);
#100528=AXIS2_PLACEMENT_3D('',#180839,#115922,#115923);
#100529=AXIS2_PLACEMENT_3D('',#180841,#115925,#115926);
#100530=AXIS2_PLACEMENT_3D('',#180845,#115928,#115929);
#100531=AXIS2_PLACEMENT_3D('',#180847,#115931,#115932);
#100532=AXIS2_PLACEMENT_3D('',#180850,#115933,#115934);
#100533=AXIS2_PLACEMENT_3D('',#180854,#115936,#115937);
#100534=AXIS2_PLACEMENT_3D('',#180856,#115939,#115940);
#100535=AXIS2_PLACEMENT_3D('',#180859,#115941,#115942);
#100536=AXIS2_PLACEMENT_3D('',#180863,#115944,#115945);
#100537=AXIS2_PLACEMENT_3D('',#180865,#115946,#115947);
#100538=AXIS2_PLACEMENT_3D('',#180867,#115948,#115949);
#100539=AXIS2_PLACEMENT_3D('',#180869,#115951,#115952);
#100540=AXIS2_PLACEMENT_3D('',#180873,#115954,#115955);
#100541=AXIS2_PLACEMENT_3D('',#180875,#115957,#115958);
#100542=AXIS2_PLACEMENT_3D('',#180876,#115959,#115960);
#100543=AXIS2_PLACEMENT_3D('',#180877,#115961,#115962);
#100544=AXIS2_PLACEMENT_3D('',#180878,#115963,#115964);
#100545=AXIS2_PLACEMENT_3D('',#180879,#115965,#115966);
#100546=AXIS2_PLACEMENT_3D('',#180880,#115967,#115968);
#100547=AXIS2_PLACEMENT_3D('',#180881,#115969,#115970);
#100548=AXIS2_PLACEMENT_3D('',#180882,#115971,#115972);
#100549=AXIS2_PLACEMENT_3D('',#180883,#115973,#115974);
#100550=AXIS2_PLACEMENT_3D('',#180884,#115975,#115976);
#100551=AXIS2_PLACEMENT_3D('',#180885,#115977,#115978);
#100552=AXIS2_PLACEMENT_3D('',#180886,#115979,#115980);
#100553=AXIS2_PLACEMENT_3D('',#180887,#115981,#115982);
#100554=AXIS2_PLACEMENT_3D('',#180890,#115983,#115984);
#100555=AXIS2_PLACEMENT_3D('',#180894,#115986,#115987);
#100556=AXIS2_PLACEMENT_3D('',#180896,#115988,#115989);
#100557=AXIS2_PLACEMENT_3D('',#180898,#115990,#115991);
#100558=AXIS2_PLACEMENT_3D('',#180900,#115993,#115994);
#100559=AXIS2_PLACEMENT_3D('',#180904,#115996,#115997);
#100560=AXIS2_PLACEMENT_3D('',#180906,#115999,#116000);
#100561=AXIS2_PLACEMENT_3D('',#180909,#116001,#116002);
#100562=AXIS2_PLACEMENT_3D('',#180913,#116004,#116005);
#100563=AXIS2_PLACEMENT_3D('',#180915,#116007,#116008);
#100564=AXIS2_PLACEMENT_3D('',#180918,#116009,#116010);
#100565=AXIS2_PLACEMENT_3D('',#180922,#116012,#116013);
#100566=AXIS2_PLACEMENT_3D('',#180924,#116014,#116015);
#100567=AXIS2_PLACEMENT_3D('',#180926,#116016,#116017);
#100568=AXIS2_PLACEMENT_3D('',#180928,#116019,#116020);
#100569=AXIS2_PLACEMENT_3D('',#180932,#116022,#116023);
#100570=AXIS2_PLACEMENT_3D('',#180934,#116025,#116026);
#100571=AXIS2_PLACEMENT_3D('',#180935,#116027,#116028);
#100572=AXIS2_PLACEMENT_3D('',#180936,#116029,#116030);
#100573=AXIS2_PLACEMENT_3D('',#180937,#116031,#116032);
#100574=AXIS2_PLACEMENT_3D('',#180938,#116033,#116034);
#100575=AXIS2_PLACEMENT_3D('',#180939,#116035,#116036);
#100576=AXIS2_PLACEMENT_3D('',#180940,#116037,#116038);
#100577=AXIS2_PLACEMENT_3D('',#180941,#116039,#116040);
#100578=AXIS2_PLACEMENT_3D('',#180942,#116041,#116042);
#100579=AXIS2_PLACEMENT_3D('',#180943,#116043,#116044);
#100580=AXIS2_PLACEMENT_3D('',#180944,#116045,#116046);
#100581=AXIS2_PLACEMENT_3D('',#180945,#116047,#116048);
#100582=AXIS2_PLACEMENT_3D('',#180946,#116049,#116050);
#100583=AXIS2_PLACEMENT_3D('',#180949,#116051,#116052);
#100584=AXIS2_PLACEMENT_3D('',#180953,#116054,#116055);
#100585=AXIS2_PLACEMENT_3D('',#180955,#116056,#116057);
#100586=AXIS2_PLACEMENT_3D('',#180957,#116058,#116059);
#100587=AXIS2_PLACEMENT_3D('',#180959,#116061,#116062);
#100588=AXIS2_PLACEMENT_3D('',#180963,#116064,#116065);
#100589=AXIS2_PLACEMENT_3D('',#180965,#116067,#116068);
#100590=AXIS2_PLACEMENT_3D('',#180968,#116069,#116070);
#100591=AXIS2_PLACEMENT_3D('',#180972,#116072,#116073);
#100592=AXIS2_PLACEMENT_3D('',#180974,#116075,#116076);
#100593=AXIS2_PLACEMENT_3D('',#180977,#116077,#116078);
#100594=AXIS2_PLACEMENT_3D('',#180981,#116080,#116081);
#100595=AXIS2_PLACEMENT_3D('',#180983,#116082,#116083);
#100596=AXIS2_PLACEMENT_3D('',#180985,#116084,#116085);
#100597=AXIS2_PLACEMENT_3D('',#180987,#116087,#116088);
#100598=AXIS2_PLACEMENT_3D('',#180991,#116090,#116091);
#100599=AXIS2_PLACEMENT_3D('',#180993,#116093,#116094);
#100600=AXIS2_PLACEMENT_3D('',#180994,#116095,#116096);
#100601=AXIS2_PLACEMENT_3D('',#180995,#116097,#116098);
#100602=AXIS2_PLACEMENT_3D('',#180996,#116099,#116100);
#100603=AXIS2_PLACEMENT_3D('',#180997,#116101,#116102);
#100604=AXIS2_PLACEMENT_3D('',#180998,#116103,#116104);
#100605=AXIS2_PLACEMENT_3D('',#180999,#116105,#116106);
#100606=AXIS2_PLACEMENT_3D('',#181000,#116107,#116108);
#100607=AXIS2_PLACEMENT_3D('',#181001,#116109,#116110);
#100608=AXIS2_PLACEMENT_3D('',#181002,#116111,#116112);
#100609=AXIS2_PLACEMENT_3D('',#181003,#116113,#116114);
#100610=AXIS2_PLACEMENT_3D('',#181004,#116115,#116116);
#100611=AXIS2_PLACEMENT_3D('',#181005,#116117,#116118);
#100612=AXIS2_PLACEMENT_3D('',#181008,#116119,#116120);
#100613=AXIS2_PLACEMENT_3D('',#181012,#116122,#116123);
#100614=AXIS2_PLACEMENT_3D('',#181014,#116124,#116125);
#100615=AXIS2_PLACEMENT_3D('',#181016,#116126,#116127);
#100616=AXIS2_PLACEMENT_3D('',#181018,#116129,#116130);
#100617=AXIS2_PLACEMENT_3D('',#181022,#116132,#116133);
#100618=AXIS2_PLACEMENT_3D('',#181024,#116135,#116136);
#100619=AXIS2_PLACEMENT_3D('',#181027,#116137,#116138);
#100620=AXIS2_PLACEMENT_3D('',#181031,#116140,#116141);
#100621=AXIS2_PLACEMENT_3D('',#181033,#116143,#116144);
#100622=AXIS2_PLACEMENT_3D('',#181036,#116145,#116146);
#100623=AXIS2_PLACEMENT_3D('',#181040,#116148,#116149);
#100624=AXIS2_PLACEMENT_3D('',#181042,#116150,#116151);
#100625=AXIS2_PLACEMENT_3D('',#181044,#116152,#116153);
#100626=AXIS2_PLACEMENT_3D('',#181046,#116155,#116156);
#100627=AXIS2_PLACEMENT_3D('',#181050,#116158,#116159);
#100628=AXIS2_PLACEMENT_3D('',#181052,#116161,#116162);
#100629=AXIS2_PLACEMENT_3D('',#181053,#116163,#116164);
#100630=AXIS2_PLACEMENT_3D('',#181054,#116165,#116166);
#100631=AXIS2_PLACEMENT_3D('',#181055,#116167,#116168);
#100632=AXIS2_PLACEMENT_3D('',#181056,#116169,#116170);
#100633=AXIS2_PLACEMENT_3D('',#181057,#116171,#116172);
#100634=AXIS2_PLACEMENT_3D('',#181058,#116173,#116174);
#100635=AXIS2_PLACEMENT_3D('',#181059,#116175,#116176);
#100636=AXIS2_PLACEMENT_3D('',#181060,#116177,#116178);
#100637=AXIS2_PLACEMENT_3D('',#181061,#116179,#116180);
#100638=AXIS2_PLACEMENT_3D('',#181062,#116181,#116182);
#100639=AXIS2_PLACEMENT_3D('',#181063,#116183,#116184);
#100640=AXIS2_PLACEMENT_3D('',#181064,#116185,#116186);
#100641=AXIS2_PLACEMENT_3D('',#181067,#116187,#116188);
#100642=AXIS2_PLACEMENT_3D('',#181071,#116190,#116191);
#100643=AXIS2_PLACEMENT_3D('',#181073,#116192,#116193);
#100644=AXIS2_PLACEMENT_3D('',#181075,#116194,#116195);
#100645=AXIS2_PLACEMENT_3D('',#181077,#116197,#116198);
#100646=AXIS2_PLACEMENT_3D('',#181081,#116200,#116201);
#100647=AXIS2_PLACEMENT_3D('',#181083,#116203,#116204);
#100648=AXIS2_PLACEMENT_3D('',#181086,#116205,#116206);
#100649=AXIS2_PLACEMENT_3D('',#181090,#116208,#116209);
#100650=AXIS2_PLACEMENT_3D('',#181092,#116211,#116212);
#100651=AXIS2_PLACEMENT_3D('',#181095,#116213,#116214);
#100652=AXIS2_PLACEMENT_3D('',#181099,#116216,#116217);
#100653=AXIS2_PLACEMENT_3D('',#181101,#116218,#116219);
#100654=AXIS2_PLACEMENT_3D('',#181103,#116220,#116221);
#100655=AXIS2_PLACEMENT_3D('',#181105,#116223,#116224);
#100656=AXIS2_PLACEMENT_3D('',#181109,#116226,#116227);
#100657=AXIS2_PLACEMENT_3D('',#181111,#116229,#116230);
#100658=AXIS2_PLACEMENT_3D('',#181112,#116231,#116232);
#100659=AXIS2_PLACEMENT_3D('',#181113,#116233,#116234);
#100660=AXIS2_PLACEMENT_3D('',#181114,#116235,#116236);
#100661=AXIS2_PLACEMENT_3D('',#181115,#116237,#116238);
#100662=AXIS2_PLACEMENT_3D('',#181116,#116239,#116240);
#100663=AXIS2_PLACEMENT_3D('',#181117,#116241,#116242);
#100664=AXIS2_PLACEMENT_3D('',#181118,#116243,#116244);
#100665=AXIS2_PLACEMENT_3D('',#181119,#116245,#116246);
#100666=AXIS2_PLACEMENT_3D('',#181120,#116247,#116248);
#100667=AXIS2_PLACEMENT_3D('',#181121,#116249,#116250);
#100668=AXIS2_PLACEMENT_3D('',#181122,#116251,#116252);
#100669=AXIS2_PLACEMENT_3D('',#181123,#116253,#116254);
#100670=AXIS2_PLACEMENT_3D('',#181126,#116255,#116256);
#100671=AXIS2_PLACEMENT_3D('',#181130,#116258,#116259);
#100672=AXIS2_PLACEMENT_3D('',#181132,#116260,#116261);
#100673=AXIS2_PLACEMENT_3D('',#181134,#116262,#116263);
#100674=AXIS2_PLACEMENT_3D('',#181136,#116265,#116266);
#100675=AXIS2_PLACEMENT_3D('',#181140,#116268,#116269);
#100676=AXIS2_PLACEMENT_3D('',#181142,#116271,#116272);
#100677=AXIS2_PLACEMENT_3D('',#181145,#116273,#116274);
#100678=AXIS2_PLACEMENT_3D('',#181149,#116276,#116277);
#100679=AXIS2_PLACEMENT_3D('',#181151,#116279,#116280);
#100680=AXIS2_PLACEMENT_3D('',#181154,#116281,#116282);
#100681=AXIS2_PLACEMENT_3D('',#181158,#116284,#116285);
#100682=AXIS2_PLACEMENT_3D('',#181160,#116286,#116287);
#100683=AXIS2_PLACEMENT_3D('',#181162,#116288,#116289);
#100684=AXIS2_PLACEMENT_3D('',#181164,#116291,#116292);
#100685=AXIS2_PLACEMENT_3D('',#181168,#116294,#116295);
#100686=AXIS2_PLACEMENT_3D('',#181170,#116297,#116298);
#100687=AXIS2_PLACEMENT_3D('',#181171,#116299,#116300);
#100688=AXIS2_PLACEMENT_3D('',#181172,#116301,#116302);
#100689=AXIS2_PLACEMENT_3D('',#181173,#116303,#116304);
#100690=AXIS2_PLACEMENT_3D('',#181174,#116305,#116306);
#100691=AXIS2_PLACEMENT_3D('',#181175,#116307,#116308);
#100692=AXIS2_PLACEMENT_3D('',#181176,#116309,#116310);
#100693=AXIS2_PLACEMENT_3D('',#181177,#116311,#116312);
#100694=AXIS2_PLACEMENT_3D('',#181178,#116313,#116314);
#100695=AXIS2_PLACEMENT_3D('',#181179,#116315,#116316);
#100696=AXIS2_PLACEMENT_3D('',#181180,#116317,#116318);
#100697=AXIS2_PLACEMENT_3D('',#181181,#116319,#116320);
#100698=AXIS2_PLACEMENT_3D('',#181182,#116321,#116322);
#100699=AXIS2_PLACEMENT_3D('',#181185,#116323,#116324);
#100700=AXIS2_PLACEMENT_3D('',#181189,#116326,#116327);
#100701=AXIS2_PLACEMENT_3D('',#181191,#116328,#116329);
#100702=AXIS2_PLACEMENT_3D('',#181193,#116330,#116331);
#100703=AXIS2_PLACEMENT_3D('',#181195,#116333,#116334);
#100704=AXIS2_PLACEMENT_3D('',#181199,#116336,#116337);
#100705=AXIS2_PLACEMENT_3D('',#181201,#116339,#116340);
#100706=AXIS2_PLACEMENT_3D('',#181204,#116341,#116342);
#100707=AXIS2_PLACEMENT_3D('',#181208,#116344,#116345);
#100708=AXIS2_PLACEMENT_3D('',#181210,#116347,#116348);
#100709=AXIS2_PLACEMENT_3D('',#181213,#116349,#116350);
#100710=AXIS2_PLACEMENT_3D('',#181217,#116352,#116353);
#100711=AXIS2_PLACEMENT_3D('',#181219,#116354,#116355);
#100712=AXIS2_PLACEMENT_3D('',#181221,#116356,#116357);
#100713=AXIS2_PLACEMENT_3D('',#181223,#116359,#116360);
#100714=AXIS2_PLACEMENT_3D('',#181227,#116362,#116363);
#100715=AXIS2_PLACEMENT_3D('',#181229,#116365,#116366);
#100716=AXIS2_PLACEMENT_3D('',#181230,#116367,#116368);
#100717=AXIS2_PLACEMENT_3D('',#181231,#116369,#116370);
#100718=AXIS2_PLACEMENT_3D('',#181232,#116371,#116372);
#100719=AXIS2_PLACEMENT_3D('',#181233,#116373,#116374);
#100720=AXIS2_PLACEMENT_3D('',#181234,#116375,#116376);
#100721=AXIS2_PLACEMENT_3D('',#181235,#116377,#116378);
#100722=AXIS2_PLACEMENT_3D('',#181236,#116379,#116380);
#100723=AXIS2_PLACEMENT_3D('',#181237,#116381,#116382);
#100724=AXIS2_PLACEMENT_3D('',#181238,#116383,#116384);
#100725=AXIS2_PLACEMENT_3D('',#181239,#116385,#116386);
#100726=AXIS2_PLACEMENT_3D('',#181240,#116387,#116388);
#100727=AXIS2_PLACEMENT_3D('',#181241,#116389,#116390);
#100728=AXIS2_PLACEMENT_3D('',#181244,#116391,#116392);
#100729=AXIS2_PLACEMENT_3D('',#181248,#116394,#116395);
#100730=AXIS2_PLACEMENT_3D('',#181250,#116396,#116397);
#100731=AXIS2_PLACEMENT_3D('',#181252,#116398,#116399);
#100732=AXIS2_PLACEMENT_3D('',#181254,#116401,#116402);
#100733=AXIS2_PLACEMENT_3D('',#181258,#116404,#116405);
#100734=AXIS2_PLACEMENT_3D('',#181260,#116407,#116408);
#100735=AXIS2_PLACEMENT_3D('',#181263,#116409,#116410);
#100736=AXIS2_PLACEMENT_3D('',#181267,#116412,#116413);
#100737=AXIS2_PLACEMENT_3D('',#181269,#116415,#116416);
#100738=AXIS2_PLACEMENT_3D('',#181272,#116417,#116418);
#100739=AXIS2_PLACEMENT_3D('',#181276,#116420,#116421);
#100740=AXIS2_PLACEMENT_3D('',#181278,#116422,#116423);
#100741=AXIS2_PLACEMENT_3D('',#181280,#116424,#116425);
#100742=AXIS2_PLACEMENT_3D('',#181282,#116427,#116428);
#100743=AXIS2_PLACEMENT_3D('',#181286,#116430,#116431);
#100744=AXIS2_PLACEMENT_3D('',#181288,#116433,#116434);
#100745=AXIS2_PLACEMENT_3D('',#181289,#116435,#116436);
#100746=AXIS2_PLACEMENT_3D('',#181290,#116437,#116438);
#100747=AXIS2_PLACEMENT_3D('',#181291,#116439,#116440);
#100748=AXIS2_PLACEMENT_3D('',#181292,#116441,#116442);
#100749=AXIS2_PLACEMENT_3D('',#181293,#116443,#116444);
#100750=AXIS2_PLACEMENT_3D('',#181294,#116445,#116446);
#100751=AXIS2_PLACEMENT_3D('',#181295,#116447,#116448);
#100752=AXIS2_PLACEMENT_3D('',#181296,#116449,#116450);
#100753=AXIS2_PLACEMENT_3D('',#181297,#116451,#116452);
#100754=AXIS2_PLACEMENT_3D('',#181298,#116453,#116454);
#100755=AXIS2_PLACEMENT_3D('',#181299,#116455,#116456);
#100756=AXIS2_PLACEMENT_3D('',#181300,#116457,#116458);
#100757=AXIS2_PLACEMENT_3D('',#181303,#116459,#116460);
#100758=AXIS2_PLACEMENT_3D('',#181307,#116462,#116463);
#100759=AXIS2_PLACEMENT_3D('',#181309,#116464,#116465);
#100760=AXIS2_PLACEMENT_3D('',#181311,#116466,#116467);
#100761=AXIS2_PLACEMENT_3D('',#181313,#116469,#116470);
#100762=AXIS2_PLACEMENT_3D('',#181317,#116472,#116473);
#100763=AXIS2_PLACEMENT_3D('',#181319,#116475,#116476);
#100764=AXIS2_PLACEMENT_3D('',#181322,#116477,#116478);
#100765=AXIS2_PLACEMENT_3D('',#181326,#116480,#116481);
#100766=AXIS2_PLACEMENT_3D('',#181328,#116483,#116484);
#100767=AXIS2_PLACEMENT_3D('',#181331,#116485,#116486);
#100768=AXIS2_PLACEMENT_3D('',#181335,#116488,#116489);
#100769=AXIS2_PLACEMENT_3D('',#181337,#116490,#116491);
#100770=AXIS2_PLACEMENT_3D('',#181339,#116492,#116493);
#100771=AXIS2_PLACEMENT_3D('',#181341,#116495,#116496);
#100772=AXIS2_PLACEMENT_3D('',#181345,#116498,#116499);
#100773=AXIS2_PLACEMENT_3D('',#181347,#116501,#116502);
#100774=AXIS2_PLACEMENT_3D('',#181348,#116503,#116504);
#100775=AXIS2_PLACEMENT_3D('',#181349,#116505,#116506);
#100776=AXIS2_PLACEMENT_3D('',#181350,#116507,#116508);
#100777=AXIS2_PLACEMENT_3D('',#181351,#116509,#116510);
#100778=AXIS2_PLACEMENT_3D('',#181352,#116511,#116512);
#100779=AXIS2_PLACEMENT_3D('',#181353,#116513,#116514);
#100780=AXIS2_PLACEMENT_3D('',#181354,#116515,#116516);
#100781=AXIS2_PLACEMENT_3D('',#181355,#116517,#116518);
#100782=AXIS2_PLACEMENT_3D('',#181356,#116519,#116520);
#100783=AXIS2_PLACEMENT_3D('',#181357,#116521,#116522);
#100784=AXIS2_PLACEMENT_3D('',#181358,#116523,#116524);
#100785=AXIS2_PLACEMENT_3D('',#181359,#116525,#116526);
#100786=AXIS2_PLACEMENT_3D('',#181362,#116527,#116528);
#100787=AXIS2_PLACEMENT_3D('',#181366,#116530,#116531);
#100788=AXIS2_PLACEMENT_3D('',#181368,#116532,#116533);
#100789=AXIS2_PLACEMENT_3D('',#181370,#116534,#116535);
#100790=AXIS2_PLACEMENT_3D('',#181372,#116537,#116538);
#100791=AXIS2_PLACEMENT_3D('',#181376,#116540,#116541);
#100792=AXIS2_PLACEMENT_3D('',#181378,#116543,#116544);
#100793=AXIS2_PLACEMENT_3D('',#181381,#116545,#116546);
#100794=AXIS2_PLACEMENT_3D('',#181385,#116548,#116549);
#100795=AXIS2_PLACEMENT_3D('',#181387,#116551,#116552);
#100796=AXIS2_PLACEMENT_3D('',#181390,#116553,#116554);
#100797=AXIS2_PLACEMENT_3D('',#181394,#116556,#116557);
#100798=AXIS2_PLACEMENT_3D('',#181396,#116558,#116559);
#100799=AXIS2_PLACEMENT_3D('',#181398,#116560,#116561);
#100800=AXIS2_PLACEMENT_3D('',#181400,#116563,#116564);
#100801=AXIS2_PLACEMENT_3D('',#181404,#116566,#116567);
#100802=AXIS2_PLACEMENT_3D('',#181406,#116569,#116570);
#100803=AXIS2_PLACEMENT_3D('',#181407,#116571,#116572);
#100804=AXIS2_PLACEMENT_3D('',#181408,#116573,#116574);
#100805=AXIS2_PLACEMENT_3D('',#181409,#116575,#116576);
#100806=AXIS2_PLACEMENT_3D('',#181410,#116577,#116578);
#100807=AXIS2_PLACEMENT_3D('',#181411,#116579,#116580);
#100808=AXIS2_PLACEMENT_3D('',#181412,#116581,#116582);
#100809=AXIS2_PLACEMENT_3D('',#181413,#116583,#116584);
#100810=AXIS2_PLACEMENT_3D('',#181414,#116585,#116586);
#100811=AXIS2_PLACEMENT_3D('',#181415,#116587,#116588);
#100812=AXIS2_PLACEMENT_3D('',#181416,#116589,#116590);
#100813=AXIS2_PLACEMENT_3D('',#181417,#116591,#116592);
#100814=AXIS2_PLACEMENT_3D('',#181418,#116593,#116594);
#100815=AXIS2_PLACEMENT_3D('',#181421,#116595,#116596);
#100816=AXIS2_PLACEMENT_3D('',#181425,#116598,#116599);
#100817=AXIS2_PLACEMENT_3D('',#181427,#116600,#116601);
#100818=AXIS2_PLACEMENT_3D('',#181429,#116602,#116603);
#100819=AXIS2_PLACEMENT_3D('',#181431,#116605,#116606);
#100820=AXIS2_PLACEMENT_3D('',#181435,#116608,#116609);
#100821=AXIS2_PLACEMENT_3D('',#181437,#116611,#116612);
#100822=AXIS2_PLACEMENT_3D('',#181440,#116613,#116614);
#100823=AXIS2_PLACEMENT_3D('',#181444,#116616,#116617);
#100824=AXIS2_PLACEMENT_3D('',#181446,#116619,#116620);
#100825=AXIS2_PLACEMENT_3D('',#181449,#116621,#116622);
#100826=AXIS2_PLACEMENT_3D('',#181453,#116624,#116625);
#100827=AXIS2_PLACEMENT_3D('',#181455,#116626,#116627);
#100828=AXIS2_PLACEMENT_3D('',#181457,#116628,#116629);
#100829=AXIS2_PLACEMENT_3D('',#181459,#116631,#116632);
#100830=AXIS2_PLACEMENT_3D('',#181463,#116634,#116635);
#100831=AXIS2_PLACEMENT_3D('',#181465,#116637,#116638);
#100832=AXIS2_PLACEMENT_3D('',#181466,#116639,#116640);
#100833=AXIS2_PLACEMENT_3D('',#181467,#116641,#116642);
#100834=AXIS2_PLACEMENT_3D('',#181468,#116643,#116644);
#100835=AXIS2_PLACEMENT_3D('',#181469,#116645,#116646);
#100836=AXIS2_PLACEMENT_3D('',#181470,#116647,#116648);
#100837=AXIS2_PLACEMENT_3D('',#181471,#116649,#116650);
#100838=AXIS2_PLACEMENT_3D('',#181472,#116651,#116652);
#100839=AXIS2_PLACEMENT_3D('',#181473,#116653,#116654);
#100840=AXIS2_PLACEMENT_3D('',#181474,#116655,#116656);
#100841=AXIS2_PLACEMENT_3D('',#181475,#116657,#116658);
#100842=AXIS2_PLACEMENT_3D('',#181476,#116659,#116660);
#100843=AXIS2_PLACEMENT_3D('',#181477,#116661,#116662);
#100844=AXIS2_PLACEMENT_3D('',#181480,#116663,#116664);
#100845=AXIS2_PLACEMENT_3D('',#181484,#116666,#116667);
#100846=AXIS2_PLACEMENT_3D('',#181486,#116668,#116669);
#100847=AXIS2_PLACEMENT_3D('',#181488,#116670,#116671);
#100848=AXIS2_PLACEMENT_3D('',#181490,#116673,#116674);
#100849=AXIS2_PLACEMENT_3D('',#181494,#116676,#116677);
#100850=AXIS2_PLACEMENT_3D('',#181496,#116679,#116680);
#100851=AXIS2_PLACEMENT_3D('',#181499,#116681,#116682);
#100852=AXIS2_PLACEMENT_3D('',#181503,#116684,#116685);
#100853=AXIS2_PLACEMENT_3D('',#181505,#116687,#116688);
#100854=AXIS2_PLACEMENT_3D('',#181508,#116689,#116690);
#100855=AXIS2_PLACEMENT_3D('',#181512,#116692,#116693);
#100856=AXIS2_PLACEMENT_3D('',#181514,#116694,#116695);
#100857=AXIS2_PLACEMENT_3D('',#181516,#116696,#116697);
#100858=AXIS2_PLACEMENT_3D('',#181518,#116699,#116700);
#100859=AXIS2_PLACEMENT_3D('',#181522,#116702,#116703);
#100860=AXIS2_PLACEMENT_3D('',#181524,#116705,#116706);
#100861=AXIS2_PLACEMENT_3D('',#181525,#116707,#116708);
#100862=AXIS2_PLACEMENT_3D('',#181526,#116709,#116710);
#100863=AXIS2_PLACEMENT_3D('',#181527,#116711,#116712);
#100864=AXIS2_PLACEMENT_3D('',#181528,#116713,#116714);
#100865=AXIS2_PLACEMENT_3D('',#181529,#116715,#116716);
#100866=AXIS2_PLACEMENT_3D('',#181530,#116717,#116718);
#100867=AXIS2_PLACEMENT_3D('',#181531,#116719,#116720);
#100868=AXIS2_PLACEMENT_3D('',#181532,#116721,#116722);
#100869=AXIS2_PLACEMENT_3D('',#181533,#116723,#116724);
#100870=AXIS2_PLACEMENT_3D('',#181534,#116725,#116726);
#100871=AXIS2_PLACEMENT_3D('',#181535,#116727,#116728);
#100872=AXIS2_PLACEMENT_3D('',#181536,#116729,#116730);
#100873=AXIS2_PLACEMENT_3D('',#181539,#116731,#116732);
#100874=AXIS2_PLACEMENT_3D('',#181543,#116734,#116735);
#100875=AXIS2_PLACEMENT_3D('',#181545,#116736,#116737);
#100876=AXIS2_PLACEMENT_3D('',#181547,#116738,#116739);
#100877=AXIS2_PLACEMENT_3D('',#181549,#116741,#116742);
#100878=AXIS2_PLACEMENT_3D('',#181553,#116744,#116745);
#100879=AXIS2_PLACEMENT_3D('',#181555,#116747,#116748);
#100880=AXIS2_PLACEMENT_3D('',#181558,#116749,#116750);
#100881=AXIS2_PLACEMENT_3D('',#181562,#116752,#116753);
#100882=AXIS2_PLACEMENT_3D('',#181564,#116755,#116756);
#100883=AXIS2_PLACEMENT_3D('',#181567,#116757,#116758);
#100884=AXIS2_PLACEMENT_3D('',#181571,#116760,#116761);
#100885=AXIS2_PLACEMENT_3D('',#181573,#116762,#116763);
#100886=AXIS2_PLACEMENT_3D('',#181575,#116764,#116765);
#100887=AXIS2_PLACEMENT_3D('',#181577,#116767,#116768);
#100888=AXIS2_PLACEMENT_3D('',#181581,#116770,#116771);
#100889=AXIS2_PLACEMENT_3D('',#181583,#116773,#116774);
#100890=AXIS2_PLACEMENT_3D('',#181584,#116775,#116776);
#100891=AXIS2_PLACEMENT_3D('',#181585,#116777,#116778);
#100892=AXIS2_PLACEMENT_3D('',#181586,#116779,#116780);
#100893=AXIS2_PLACEMENT_3D('',#181587,#116781,#116782);
#100894=AXIS2_PLACEMENT_3D('',#181588,#116783,#116784);
#100895=AXIS2_PLACEMENT_3D('',#181589,#116785,#116786);
#100896=AXIS2_PLACEMENT_3D('',#181590,#116787,#116788);
#100897=AXIS2_PLACEMENT_3D('',#181591,#116789,#116790);
#100898=AXIS2_PLACEMENT_3D('',#181592,#116791,#116792);
#100899=AXIS2_PLACEMENT_3D('',#181593,#116793,#116794);
#100900=AXIS2_PLACEMENT_3D('',#181594,#116795,#116796);
#100901=AXIS2_PLACEMENT_3D('',#181595,#116797,#116798);
#100902=AXIS2_PLACEMENT_3D('',#181598,#116799,#116800);
#100903=AXIS2_PLACEMENT_3D('',#181602,#116802,#116803);
#100904=AXIS2_PLACEMENT_3D('',#181604,#116804,#116805);
#100905=AXIS2_PLACEMENT_3D('',#181606,#116806,#116807);
#100906=AXIS2_PLACEMENT_3D('',#181608,#116809,#116810);
#100907=AXIS2_PLACEMENT_3D('',#181612,#116812,#116813);
#100908=AXIS2_PLACEMENT_3D('',#181614,#116815,#116816);
#100909=AXIS2_PLACEMENT_3D('',#181617,#116817,#116818);
#100910=AXIS2_PLACEMENT_3D('',#181621,#116820,#116821);
#100911=AXIS2_PLACEMENT_3D('',#181623,#116823,#116824);
#100912=AXIS2_PLACEMENT_3D('',#181626,#116825,#116826);
#100913=AXIS2_PLACEMENT_3D('',#181630,#116828,#116829);
#100914=AXIS2_PLACEMENT_3D('',#181632,#116830,#116831);
#100915=AXIS2_PLACEMENT_3D('',#181634,#116832,#116833);
#100916=AXIS2_PLACEMENT_3D('',#181636,#116835,#116836);
#100917=AXIS2_PLACEMENT_3D('',#181640,#116838,#116839);
#100918=AXIS2_PLACEMENT_3D('',#181642,#116841,#116842);
#100919=AXIS2_PLACEMENT_3D('',#181643,#116843,#116844);
#100920=AXIS2_PLACEMENT_3D('',#181644,#116845,#116846);
#100921=AXIS2_PLACEMENT_3D('',#181645,#116847,#116848);
#100922=AXIS2_PLACEMENT_3D('',#181646,#116849,#116850);
#100923=AXIS2_PLACEMENT_3D('',#181647,#116851,#116852);
#100924=AXIS2_PLACEMENT_3D('',#181648,#116853,#116854);
#100925=AXIS2_PLACEMENT_3D('',#181649,#116855,#116856);
#100926=AXIS2_PLACEMENT_3D('',#181650,#116857,#116858);
#100927=AXIS2_PLACEMENT_3D('',#181651,#116859,#116860);
#100928=AXIS2_PLACEMENT_3D('',#181652,#116861,#116862);
#100929=AXIS2_PLACEMENT_3D('',#181653,#116863,#116864);
#100930=AXIS2_PLACEMENT_3D('',#181654,#116865,#116866);
#100931=AXIS2_PLACEMENT_3D('',#181657,#116867,#116868);
#100932=AXIS2_PLACEMENT_3D('',#181661,#116870,#116871);
#100933=AXIS2_PLACEMENT_3D('',#181663,#116872,#116873);
#100934=AXIS2_PLACEMENT_3D('',#181665,#116874,#116875);
#100935=AXIS2_PLACEMENT_3D('',#181667,#116877,#116878);
#100936=AXIS2_PLACEMENT_3D('',#181671,#116880,#116881);
#100937=AXIS2_PLACEMENT_3D('',#181673,#116883,#116884);
#100938=AXIS2_PLACEMENT_3D('',#181676,#116885,#116886);
#100939=AXIS2_PLACEMENT_3D('',#181680,#116888,#116889);
#100940=AXIS2_PLACEMENT_3D('',#181682,#116891,#116892);
#100941=AXIS2_PLACEMENT_3D('',#181685,#116893,#116894);
#100942=AXIS2_PLACEMENT_3D('',#181689,#116896,#116897);
#100943=AXIS2_PLACEMENT_3D('',#181691,#116898,#116899);
#100944=AXIS2_PLACEMENT_3D('',#181693,#116900,#116901);
#100945=AXIS2_PLACEMENT_3D('',#181695,#116903,#116904);
#100946=AXIS2_PLACEMENT_3D('',#181699,#116906,#116907);
#100947=AXIS2_PLACEMENT_3D('',#181701,#116909,#116910);
#100948=AXIS2_PLACEMENT_3D('',#181702,#116911,#116912);
#100949=AXIS2_PLACEMENT_3D('',#181703,#116913,#116914);
#100950=AXIS2_PLACEMENT_3D('',#181704,#116915,#116916);
#100951=AXIS2_PLACEMENT_3D('',#181705,#116917,#116918);
#100952=AXIS2_PLACEMENT_3D('',#181706,#116919,#116920);
#100953=AXIS2_PLACEMENT_3D('',#181707,#116921,#116922);
#100954=AXIS2_PLACEMENT_3D('',#181708,#116923,#116924);
#100955=AXIS2_PLACEMENT_3D('',#181709,#116925,#116926);
#100956=AXIS2_PLACEMENT_3D('',#181710,#116927,#116928);
#100957=AXIS2_PLACEMENT_3D('',#181711,#116929,#116930);
#100958=AXIS2_PLACEMENT_3D('',#181712,#116931,#116932);
#100959=AXIS2_PLACEMENT_3D('',#181713,#116933,#116934);
#100960=AXIS2_PLACEMENT_3D('',#181716,#116935,#116936);
#100961=AXIS2_PLACEMENT_3D('',#181720,#116938,#116939);
#100962=AXIS2_PLACEMENT_3D('',#181722,#116940,#116941);
#100963=AXIS2_PLACEMENT_3D('',#181724,#116942,#116943);
#100964=AXIS2_PLACEMENT_3D('',#181726,#116945,#116946);
#100965=AXIS2_PLACEMENT_3D('',#181730,#116948,#116949);
#100966=AXIS2_PLACEMENT_3D('',#181732,#116951,#116952);
#100967=AXIS2_PLACEMENT_3D('',#181735,#116953,#116954);
#100968=AXIS2_PLACEMENT_3D('',#181739,#116956,#116957);
#100969=AXIS2_PLACEMENT_3D('',#181741,#116959,#116960);
#100970=AXIS2_PLACEMENT_3D('',#181744,#116961,#116962);
#100971=AXIS2_PLACEMENT_3D('',#181748,#116964,#116965);
#100972=AXIS2_PLACEMENT_3D('',#181750,#116966,#116967);
#100973=AXIS2_PLACEMENT_3D('',#181752,#116968,#116969);
#100974=AXIS2_PLACEMENT_3D('',#181754,#116971,#116972);
#100975=AXIS2_PLACEMENT_3D('',#181758,#116974,#116975);
#100976=AXIS2_PLACEMENT_3D('',#181760,#116977,#116978);
#100977=AXIS2_PLACEMENT_3D('',#181761,#116979,#116980);
#100978=AXIS2_PLACEMENT_3D('',#181762,#116981,#116982);
#100979=AXIS2_PLACEMENT_3D('',#181763,#116983,#116984);
#100980=AXIS2_PLACEMENT_3D('',#181764,#116985,#116986);
#100981=AXIS2_PLACEMENT_3D('',#181765,#116987,#116988);
#100982=AXIS2_PLACEMENT_3D('',#181766,#116989,#116990);
#100983=AXIS2_PLACEMENT_3D('',#181767,#116991,#116992);
#100984=AXIS2_PLACEMENT_3D('',#181768,#116993,#116994);
#100985=AXIS2_PLACEMENT_3D('',#181769,#116995,#116996);
#100986=AXIS2_PLACEMENT_3D('',#181770,#116997,#116998);
#100987=AXIS2_PLACEMENT_3D('',#181771,#116999,#117000);
#100988=AXIS2_PLACEMENT_3D('',#181772,#117001,#117002);
#100989=AXIS2_PLACEMENT_3D('',#181775,#117003,#117004);
#100990=AXIS2_PLACEMENT_3D('',#181779,#117006,#117007);
#100991=AXIS2_PLACEMENT_3D('',#181781,#117008,#117009);
#100992=AXIS2_PLACEMENT_3D('',#181783,#117010,#117011);
#100993=AXIS2_PLACEMENT_3D('',#181785,#117013,#117014);
#100994=AXIS2_PLACEMENT_3D('',#181789,#117016,#117017);
#100995=AXIS2_PLACEMENT_3D('',#181791,#117019,#117020);
#100996=AXIS2_PLACEMENT_3D('',#181794,#117021,#117022);
#100997=AXIS2_PLACEMENT_3D('',#181798,#117024,#117025);
#100998=AXIS2_PLACEMENT_3D('',#181800,#117027,#117028);
#100999=AXIS2_PLACEMENT_3D('',#181803,#117029,#117030);
#101000=AXIS2_PLACEMENT_3D('',#181807,#117032,#117033);
#101001=AXIS2_PLACEMENT_3D('',#181809,#117034,#117035);
#101002=AXIS2_PLACEMENT_3D('',#181811,#117036,#117037);
#101003=AXIS2_PLACEMENT_3D('',#181813,#117039,#117040);
#101004=AXIS2_PLACEMENT_3D('',#181817,#117042,#117043);
#101005=AXIS2_PLACEMENT_3D('',#181819,#117045,#117046);
#101006=AXIS2_PLACEMENT_3D('',#181820,#117047,#117048);
#101007=AXIS2_PLACEMENT_3D('',#181821,#117049,#117050);
#101008=AXIS2_PLACEMENT_3D('',#181822,#117051,#117052);
#101009=AXIS2_PLACEMENT_3D('',#181823,#117053,#117054);
#101010=AXIS2_PLACEMENT_3D('',#181824,#117055,#117056);
#101011=AXIS2_PLACEMENT_3D('',#181825,#117057,#117058);
#101012=AXIS2_PLACEMENT_3D('',#181826,#117059,#117060);
#101013=AXIS2_PLACEMENT_3D('',#181827,#117061,#117062);
#101014=AXIS2_PLACEMENT_3D('',#181828,#117063,#117064);
#101015=AXIS2_PLACEMENT_3D('',#181829,#117065,#117066);
#101016=AXIS2_PLACEMENT_3D('',#181830,#117067,#117068);
#101017=AXIS2_PLACEMENT_3D('',#181831,#117069,#117070);
#101018=AXIS2_PLACEMENT_3D('',#181834,#117071,#117072);
#101019=AXIS2_PLACEMENT_3D('',#181838,#117074,#117075);
#101020=AXIS2_PLACEMENT_3D('',#181840,#117076,#117077);
#101021=AXIS2_PLACEMENT_3D('',#181842,#117078,#117079);
#101022=AXIS2_PLACEMENT_3D('',#181844,#117081,#117082);
#101023=AXIS2_PLACEMENT_3D('',#181848,#117084,#117085);
#101024=AXIS2_PLACEMENT_3D('',#181850,#117087,#117088);
#101025=AXIS2_PLACEMENT_3D('',#181853,#117089,#117090);
#101026=AXIS2_PLACEMENT_3D('',#181857,#117092,#117093);
#101027=AXIS2_PLACEMENT_3D('',#181859,#117095,#117096);
#101028=AXIS2_PLACEMENT_3D('',#181862,#117097,#117098);
#101029=AXIS2_PLACEMENT_3D('',#181866,#117100,#117101);
#101030=AXIS2_PLACEMENT_3D('',#181868,#117102,#117103);
#101031=AXIS2_PLACEMENT_3D('',#181870,#117104,#117105);
#101032=AXIS2_PLACEMENT_3D('',#181872,#117107,#117108);
#101033=AXIS2_PLACEMENT_3D('',#181876,#117110,#117111);
#101034=AXIS2_PLACEMENT_3D('',#181878,#117113,#117114);
#101035=AXIS2_PLACEMENT_3D('',#181879,#117115,#117116);
#101036=AXIS2_PLACEMENT_3D('',#181880,#117117,#117118);
#101037=AXIS2_PLACEMENT_3D('',#181881,#117119,#117120);
#101038=AXIS2_PLACEMENT_3D('',#181882,#117121,#117122);
#101039=AXIS2_PLACEMENT_3D('',#181883,#117123,#117124);
#101040=AXIS2_PLACEMENT_3D('',#181884,#117125,#117126);
#101041=AXIS2_PLACEMENT_3D('',#181885,#117127,#117128);
#101042=AXIS2_PLACEMENT_3D('',#181886,#117129,#117130);
#101043=AXIS2_PLACEMENT_3D('',#181887,#117131,#117132);
#101044=AXIS2_PLACEMENT_3D('',#181888,#117133,#117134);
#101045=AXIS2_PLACEMENT_3D('',#181889,#117135,#117136);
#101046=AXIS2_PLACEMENT_3D('',#181890,#117137,#117138);
#101047=AXIS2_PLACEMENT_3D('',#181893,#117139,#117140);
#101048=AXIS2_PLACEMENT_3D('',#181897,#117142,#117143);
#101049=AXIS2_PLACEMENT_3D('',#181899,#117144,#117145);
#101050=AXIS2_PLACEMENT_3D('',#181901,#117146,#117147);
#101051=AXIS2_PLACEMENT_3D('',#181903,#117149,#117150);
#101052=AXIS2_PLACEMENT_3D('',#181907,#117152,#117153);
#101053=AXIS2_PLACEMENT_3D('',#181909,#117155,#117156);
#101054=AXIS2_PLACEMENT_3D('',#181912,#117157,#117158);
#101055=AXIS2_PLACEMENT_3D('',#181916,#117160,#117161);
#101056=AXIS2_PLACEMENT_3D('',#181918,#117163,#117164);
#101057=AXIS2_PLACEMENT_3D('',#181921,#117165,#117166);
#101058=AXIS2_PLACEMENT_3D('',#181925,#117168,#117169);
#101059=AXIS2_PLACEMENT_3D('',#181927,#117170,#117171);
#101060=AXIS2_PLACEMENT_3D('',#181929,#117172,#117173);
#101061=AXIS2_PLACEMENT_3D('',#181931,#117175,#117176);
#101062=AXIS2_PLACEMENT_3D('',#181935,#117178,#117179);
#101063=AXIS2_PLACEMENT_3D('',#181937,#117181,#117182);
#101064=AXIS2_PLACEMENT_3D('',#181938,#117183,#117184);
#101065=AXIS2_PLACEMENT_3D('',#181939,#117185,#117186);
#101066=AXIS2_PLACEMENT_3D('',#181940,#117187,#117188);
#101067=AXIS2_PLACEMENT_3D('',#181941,#117189,#117190);
#101068=AXIS2_PLACEMENT_3D('',#181942,#117191,#117192);
#101069=AXIS2_PLACEMENT_3D('',#181943,#117193,#117194);
#101070=AXIS2_PLACEMENT_3D('',#181944,#117195,#117196);
#101071=AXIS2_PLACEMENT_3D('',#181945,#117197,#117198);
#101072=AXIS2_PLACEMENT_3D('',#181946,#117199,#117200);
#101073=AXIS2_PLACEMENT_3D('',#181947,#117201,#117202);
#101074=AXIS2_PLACEMENT_3D('',#181948,#117203,#117204);
#101075=AXIS2_PLACEMENT_3D('',#181949,#117205,#117206);
#101076=AXIS2_PLACEMENT_3D('',#181950,#117207,#117208);
#101077=AXIS2_PLACEMENT_3D('',#181953,#117209,#117210);
#101078=AXIS2_PLACEMENT_3D('',#181957,#117212,#117213);
#101079=AXIS2_PLACEMENT_3D('',#181959,#117214,#117215);
#101080=AXIS2_PLACEMENT_3D('',#181961,#117216,#117217);
#101081=AXIS2_PLACEMENT_3D('',#181963,#117219,#117220);
#101082=AXIS2_PLACEMENT_3D('',#181967,#117222,#117223);
#101083=AXIS2_PLACEMENT_3D('',#181969,#117225,#117226);
#101084=AXIS2_PLACEMENT_3D('',#181972,#117227,#117228);
#101085=AXIS2_PLACEMENT_3D('',#181976,#117230,#117231);
#101086=AXIS2_PLACEMENT_3D('',#181978,#117233,#117234);
#101087=AXIS2_PLACEMENT_3D('',#181981,#117235,#117236);
#101088=AXIS2_PLACEMENT_3D('',#181985,#117238,#117239);
#101089=AXIS2_PLACEMENT_3D('',#181987,#117240,#117241);
#101090=AXIS2_PLACEMENT_3D('',#181989,#117242,#117243);
#101091=AXIS2_PLACEMENT_3D('',#181991,#117245,#117246);
#101092=AXIS2_PLACEMENT_3D('',#181995,#117248,#117249);
#101093=AXIS2_PLACEMENT_3D('',#181997,#117251,#117252);
#101094=AXIS2_PLACEMENT_3D('',#181998,#117253,#117254);
#101095=AXIS2_PLACEMENT_3D('',#181999,#117255,#117256);
#101096=AXIS2_PLACEMENT_3D('',#182000,#117257,#117258);
#101097=AXIS2_PLACEMENT_3D('',#182001,#117259,#117260);
#101098=AXIS2_PLACEMENT_3D('',#182002,#117261,#117262);
#101099=AXIS2_PLACEMENT_3D('',#182003,#117263,#117264);
#101100=AXIS2_PLACEMENT_3D('',#182004,#117265,#117266);
#101101=AXIS2_PLACEMENT_3D('',#182005,#117267,#117268);
#101102=AXIS2_PLACEMENT_3D('',#182006,#117269,#117270);
#101103=AXIS2_PLACEMENT_3D('',#182007,#117271,#117272);
#101104=AXIS2_PLACEMENT_3D('',#182008,#117273,#117274);
#101105=AXIS2_PLACEMENT_3D('',#182009,#117275,#117276);
#101106=AXIS2_PLACEMENT_3D('',#182010,#117277,#117278);
#101107=AXIS2_PLACEMENT_3D('',#182011,#117279,#117280);
#101108=AXIS2_PLACEMENT_3D('',#182016,#117282,#117283);
#101109=AXIS2_PLACEMENT_3D('',#182019,#117285,#117286);
#101110=AXIS2_PLACEMENT_3D('',#182020,#117287,#117288);
#101111=AXIS2_PLACEMENT_3D('',#182023,#117289,#117290);
#101112=AXIS2_PLACEMENT_3D('',#182031,#117294,#117295);
#101113=AXIS2_PLACEMENT_3D('',#182037,#117298,#117299);
#101114=AXIS2_PLACEMENT_3D('',#182041,#117301,#117302);
#101115=AXIS2_PLACEMENT_3D('',#182045,#117305,#117306);
#101116=AXIS2_PLACEMENT_3D('',#182048,#117307,#117308);
#101117=AXIS2_PLACEMENT_3D('',#182056,#117312,#117313);
#101118=AXIS2_PLACEMENT_3D('',#182062,#117316,#117317);
#101119=AXIS2_PLACEMENT_3D('',#182066,#117319,#117320);
#101120=AXIS2_PLACEMENT_3D('',#182070,#117323,#117324);
#101121=AXIS2_PLACEMENT_3D('',#182175,#117325,#117326);
#101122=AXIS2_PLACEMENT_3D('',#182274,#117327,#117328);
#101123=AXIS2_PLACEMENT_3D('',#182275,#117329,#117330);
#101124=AXIS2_PLACEMENT_3D('',#182276,#117331,#117332);
#101125=AXIS2_PLACEMENT_3D('',#182289,#117333,#117334);
#101126=AXIS2_PLACEMENT_3D('',#182290,#117335,#117336);
#101127=AXIS2_PLACEMENT_3D('',#182291,#117337,#117338);
#101128=AXIS2_PLACEMENT_3D('',#182292,#117339,#117340);
#101129=AXIS2_PLACEMENT_3D('',#182293,#117341,#117342);
#101130=AXIS2_PLACEMENT_3D('',#182306,#117343,#117344);
#101131=AXIS2_PLACEMENT_3D('',#182319,#117345,#117346);
#101132=AXIS2_PLACEMENT_3D('',#182320,#117347,#117348);
#101133=AXIS2_PLACEMENT_3D('',#182321,#117349,#117350);
#101134=AXIS2_PLACEMENT_3D('',#182322,#117351,#117352);
#101135=AXIS2_PLACEMENT_3D('',#182323,#117353,#117354);
#101136=AXIS2_PLACEMENT_3D('',#182342,#117355,#117356);
#101137=AXIS2_PLACEMENT_3D('',#182343,#117357,#117358);
#101138=AXIS2_PLACEMENT_3D('',#182344,#117359,#117360);
#101139=AXIS2_PLACEMENT_3D('',#182345,#117361,#117362);
#101140=AXIS2_PLACEMENT_3D('',#182346,#117363,#117364);
#101141=AXIS2_PLACEMENT_3D('',#182359,#117365,#117366);
#101142=AXIS2_PLACEMENT_3D('',#182378,#117367,#117368);
#101143=AXIS2_PLACEMENT_3D('',#182379,#117369,#117370);
#101144=AXIS2_PLACEMENT_3D('',#182380,#117371,#117372);
#101145=AXIS2_PLACEMENT_3D('',#182381,#117373,#117374);
#101146=AXIS2_PLACEMENT_3D('',#182382,#117375,#117376);
#101147=AXIS2_PLACEMENT_3D('',#182401,#117377,#117378);
#101148=AXIS2_PLACEMENT_3D('',#182414,#117379,#117380);
#101149=AXIS2_PLACEMENT_3D('',#182415,#117381,#117382);
#101150=AXIS2_PLACEMENT_3D('',#182416,#117383,#117384);
#101151=AXIS2_PLACEMENT_3D('',#182417,#117385,#117386);
#101152=AXIS2_PLACEMENT_3D('',#182418,#117387,#117388);
#101153=AXIS2_PLACEMENT_3D('',#182437,#117389,#117390);
#101154=AXIS2_PLACEMENT_3D('',#182438,#117391,#117392);
#101155=AXIS2_PLACEMENT_3D('',#182439,#117393,#117394);
#101156=AXIS2_PLACEMENT_3D('',#182440,#117395,#117396);
#101157=AXIS2_PLACEMENT_3D('',#182441,#117397,#117398);
#101158=AXIS2_PLACEMENT_3D('',#182454,#117399,#117400);
#101159=AXIS2_PLACEMENT_3D('',#182467,#117401,#117402);
#101160=AXIS2_PLACEMENT_3D('',#182468,#117403,#117404);
#101161=AXIS2_PLACEMENT_3D('',#182469,#117405,#117406);
#101162=AXIS2_PLACEMENT_3D('',#182470,#117407,#117408);
#101163=AXIS2_PLACEMENT_3D('',#182471,#117409,#117410);
#101164=AXIS2_PLACEMENT_3D('',#182484,#117411,#117412);
#101165=AXIS2_PLACEMENT_3D('',#182485,#117413,#117414);
#101166=AXIS2_PLACEMENT_3D('',#182486,#117415,#117416);
#101167=AXIS2_PLACEMENT_3D('',#182491,#117418,#117419);
#101168=AXIS2_PLACEMENT_3D('',#182494,#117421,#117422);
#101169=AXIS2_PLACEMENT_3D('',#182495,#117423,#117424);
#101170=AXIS2_PLACEMENT_3D('',#182498,#117425,#117426);
#101171=AXIS2_PLACEMENT_3D('',#182506,#117430,#117431);
#101172=AXIS2_PLACEMENT_3D('',#182512,#117434,#117435);
#101173=AXIS2_PLACEMENT_3D('',#182516,#117437,#117438);
#101174=AXIS2_PLACEMENT_3D('',#182520,#117441,#117442);
#101175=AXIS2_PLACEMENT_3D('',#182523,#117443,#117444);
#101176=AXIS2_PLACEMENT_3D('',#182531,#117448,#117449);
#101177=AXIS2_PLACEMENT_3D('',#182537,#117452,#117453);
#101178=AXIS2_PLACEMENT_3D('',#182541,#117455,#117456);
#101179=AXIS2_PLACEMENT_3D('',#182545,#117459,#117460);
#101180=AXIS2_PLACEMENT_3D('',#182550,#117462,#117463);
#101181=AXIS2_PLACEMENT_3D('',#182553,#117465,#117466);
#101182=AXIS2_PLACEMENT_3D('',#182554,#117467,#117468);
#101183=AXIS2_PLACEMENT_3D('',#182557,#117469,#117470);
#101184=AXIS2_PLACEMENT_3D('',#182565,#117474,#117475);
#101185=AXIS2_PLACEMENT_3D('',#182571,#117478,#117479);
#101186=AXIS2_PLACEMENT_3D('',#182575,#117481,#117482);
#101187=AXIS2_PLACEMENT_3D('',#182579,#117485,#117486);
#101188=AXIS2_PLACEMENT_3D('',#182582,#117487,#117488);
#101189=AXIS2_PLACEMENT_3D('',#182590,#117492,#117493);
#101190=AXIS2_PLACEMENT_3D('',#182596,#117496,#117497);
#101191=AXIS2_PLACEMENT_3D('',#182600,#117499,#117500);
#101192=AXIS2_PLACEMENT_3D('',#182604,#117503,#117504);
#101193=AXIS2_PLACEMENT_3D('',#182609,#117506,#117507);
#101194=AXIS2_PLACEMENT_3D('',#182612,#117509,#117510);
#101195=AXIS2_PLACEMENT_3D('',#182613,#117511,#117512);
#101196=AXIS2_PLACEMENT_3D('',#182616,#117513,#117514);
#101197=AXIS2_PLACEMENT_3D('',#182624,#117518,#117519);
#101198=AXIS2_PLACEMENT_3D('',#182630,#117522,#117523);
#101199=AXIS2_PLACEMENT_3D('',#182634,#117525,#117526);
#101200=AXIS2_PLACEMENT_3D('',#182638,#117529,#117530);
#101201=AXIS2_PLACEMENT_3D('',#182641,#117531,#117532);
#101202=AXIS2_PLACEMENT_3D('',#182649,#117536,#117537);
#101203=AXIS2_PLACEMENT_3D('',#182655,#117540,#117541);
#101204=AXIS2_PLACEMENT_3D('',#182659,#117543,#117544);
#101205=AXIS2_PLACEMENT_3D('',#182663,#117547,#117548);
#101206=AXIS2_PLACEMENT_3D('',#182668,#117550,#117551);
#101207=AXIS2_PLACEMENT_3D('',#182671,#117553,#117554);
#101208=AXIS2_PLACEMENT_3D('',#182672,#117555,#117556);
#101209=AXIS2_PLACEMENT_3D('',#182675,#117557,#117558);
#101210=AXIS2_PLACEMENT_3D('',#182683,#117562,#117563);
#101211=AXIS2_PLACEMENT_3D('',#182689,#117566,#117567);
#101212=AXIS2_PLACEMENT_3D('',#182693,#117569,#117570);
#101213=AXIS2_PLACEMENT_3D('',#182697,#117573,#117574);
#101214=AXIS2_PLACEMENT_3D('',#182700,#117575,#117576);
#101215=AXIS2_PLACEMENT_3D('',#182708,#117580,#117581);
#101216=AXIS2_PLACEMENT_3D('',#182714,#117584,#117585);
#101217=AXIS2_PLACEMENT_3D('',#182718,#117587,#117588);
#101218=AXIS2_PLACEMENT_3D('',#182722,#117591,#117592);
#101219=AXIS2_PLACEMENT_3D('',#182727,#117594,#117595);
#101220=AXIS2_PLACEMENT_3D('',#182730,#117597,#117598);
#101221=AXIS2_PLACEMENT_3D('',#182731,#117599,#117600);
#101222=AXIS2_PLACEMENT_3D('',#182734,#117601,#117602);
#101223=AXIS2_PLACEMENT_3D('',#182742,#117606,#117607);
#101224=AXIS2_PLACEMENT_3D('',#182748,#117610,#117611);
#101225=AXIS2_PLACEMENT_3D('',#182752,#117613,#117614);
#101226=AXIS2_PLACEMENT_3D('',#182756,#117617,#117618);
#101227=AXIS2_PLACEMENT_3D('',#182759,#117619,#117620);
#101228=AXIS2_PLACEMENT_3D('',#182767,#117624,#117625);
#101229=AXIS2_PLACEMENT_3D('',#182773,#117628,#117629);
#101230=AXIS2_PLACEMENT_3D('',#182777,#117631,#117632);
#101231=AXIS2_PLACEMENT_3D('',#182781,#117635,#117636);
#101232=AXIS2_PLACEMENT_3D('',#182786,#117638,#117639);
#101233=AXIS2_PLACEMENT_3D('',#182789,#117641,#117642);
#101234=AXIS2_PLACEMENT_3D('',#182790,#117643,#117644);
#101235=AXIS2_PLACEMENT_3D('',#182793,#117645,#117646);
#101236=AXIS2_PLACEMENT_3D('',#182801,#117650,#117651);
#101237=AXIS2_PLACEMENT_3D('',#182807,#117654,#117655);
#101238=AXIS2_PLACEMENT_3D('',#182811,#117657,#117658);
#101239=AXIS2_PLACEMENT_3D('',#182815,#117661,#117662);
#101240=AXIS2_PLACEMENT_3D('',#182818,#117663,#117664);
#101241=AXIS2_PLACEMENT_3D('',#182826,#117668,#117669);
#101242=AXIS2_PLACEMENT_3D('',#182832,#117672,#117673);
#101243=AXIS2_PLACEMENT_3D('',#182836,#117675,#117676);
#101244=AXIS2_PLACEMENT_3D('',#182840,#117679,#117680);
#101245=AXIS2_PLACEMENT_3D('',#182845,#117682,#117683);
#101246=AXIS2_PLACEMENT_3D('',#182848,#117685,#117686);
#101247=AXIS2_PLACEMENT_3D('',#182849,#117687,#117688);
#101248=AXIS2_PLACEMENT_3D('',#182852,#117689,#117690);
#101249=AXIS2_PLACEMENT_3D('',#182860,#117694,#117695);
#101250=AXIS2_PLACEMENT_3D('',#182866,#117698,#117699);
#101251=AXIS2_PLACEMENT_3D('',#182870,#117701,#117702);
#101252=AXIS2_PLACEMENT_3D('',#182874,#117705,#117706);
#101253=AXIS2_PLACEMENT_3D('',#182877,#117707,#117708);
#101254=AXIS2_PLACEMENT_3D('',#182885,#117712,#117713);
#101255=AXIS2_PLACEMENT_3D('',#182891,#117716,#117717);
#101256=AXIS2_PLACEMENT_3D('',#182895,#117719,#117720);
#101257=AXIS2_PLACEMENT_3D('',#182899,#117723,#117724);
#101258=AXIS2_PLACEMENT_3D('',#182904,#117726,#117727);
#101259=AXIS2_PLACEMENT_3D('',#182907,#117729,#117730);
#101260=AXIS2_PLACEMENT_3D('',#182908,#117731,#117732);
#101261=AXIS2_PLACEMENT_3D('',#182911,#117733,#117734);
#101262=AXIS2_PLACEMENT_3D('',#182919,#117738,#117739);
#101263=AXIS2_PLACEMENT_3D('',#182925,#117742,#117743);
#101264=AXIS2_PLACEMENT_3D('',#182929,#117745,#117746);
#101265=AXIS2_PLACEMENT_3D('',#182933,#117749,#117750);
#101266=AXIS2_PLACEMENT_3D('',#182936,#117751,#117752);
#101267=AXIS2_PLACEMENT_3D('',#182944,#117756,#117757);
#101268=AXIS2_PLACEMENT_3D('',#182950,#117760,#117761);
#101269=AXIS2_PLACEMENT_3D('',#182954,#117763,#117764);
#101270=AXIS2_PLACEMENT_3D('',#182958,#117767,#117768);
#101271=AXIS2_PLACEMENT_3D('',#182963,#117770,#117771);
#101272=AXIS2_PLACEMENT_3D('',#182966,#117773,#117774);
#101273=AXIS2_PLACEMENT_3D('',#182967,#117775,#117776);
#101274=AXIS2_PLACEMENT_3D('',#182970,#117777,#117778);
#101275=AXIS2_PLACEMENT_3D('',#182978,#117782,#117783);
#101276=AXIS2_PLACEMENT_3D('',#182984,#117786,#117787);
#101277=AXIS2_PLACEMENT_3D('',#182988,#117789,#117790);
#101278=AXIS2_PLACEMENT_3D('',#182992,#117793,#117794);
#101279=AXIS2_PLACEMENT_3D('',#182995,#117795,#117796);
#101280=AXIS2_PLACEMENT_3D('',#183003,#117800,#117801);
#101281=AXIS2_PLACEMENT_3D('',#183009,#117804,#117805);
#101282=AXIS2_PLACEMENT_3D('',#183013,#117807,#117808);
#101283=AXIS2_PLACEMENT_3D('',#183017,#117811,#117812);
#101284=AXIS2_PLACEMENT_3D('',#183022,#117814,#117815);
#101285=AXIS2_PLACEMENT_3D('',#183025,#117817,#117818);
#101286=AXIS2_PLACEMENT_3D('',#183026,#117819,#117820);
#101287=AXIS2_PLACEMENT_3D('',#183029,#117821,#117822);
#101288=AXIS2_PLACEMENT_3D('',#183037,#117826,#117827);
#101289=AXIS2_PLACEMENT_3D('',#183043,#117830,#117831);
#101290=AXIS2_PLACEMENT_3D('',#183047,#117833,#117834);
#101291=AXIS2_PLACEMENT_3D('',#183051,#117837,#117838);
#101292=AXIS2_PLACEMENT_3D('',#183054,#117839,#117840);
#101293=AXIS2_PLACEMENT_3D('',#183062,#117844,#117845);
#101294=AXIS2_PLACEMENT_3D('',#183068,#117848,#117849);
#101295=AXIS2_PLACEMENT_3D('',#183072,#117851,#117852);
#101296=AXIS2_PLACEMENT_3D('',#183076,#117855,#117856);
#101297=AXIS2_PLACEMENT_3D('',#183081,#117858,#117859);
#101298=AXIS2_PLACEMENT_3D('',#183084,#117861,#117862);
#101299=AXIS2_PLACEMENT_3D('',#183085,#117863,#117864);
#101300=AXIS2_PLACEMENT_3D('',#183088,#117865,#117866);
#101301=AXIS2_PLACEMENT_3D('',#183096,#117870,#117871);
#101302=AXIS2_PLACEMENT_3D('',#183102,#117874,#117875);
#101303=AXIS2_PLACEMENT_3D('',#183106,#117877,#117878);
#101304=AXIS2_PLACEMENT_3D('',#183110,#117881,#117882);
#101305=AXIS2_PLACEMENT_3D('',#183113,#117883,#117884);
#101306=AXIS2_PLACEMENT_3D('',#183121,#117888,#117889);
#101307=AXIS2_PLACEMENT_3D('',#183127,#117892,#117893);
#101308=AXIS2_PLACEMENT_3D('',#183131,#117895,#117896);
#101309=AXIS2_PLACEMENT_3D('',#183135,#117899,#117900);
#101310=AXIS2_PLACEMENT_3D('',#183140,#117902,#117903);
#101311=AXIS2_PLACEMENT_3D('',#183143,#117905,#117906);
#101312=AXIS2_PLACEMENT_3D('',#183144,#117907,#117908);
#101313=AXIS2_PLACEMENT_3D('',#183147,#117909,#117910);
#101314=AXIS2_PLACEMENT_3D('',#183155,#117914,#117915);
#101315=AXIS2_PLACEMENT_3D('',#183161,#117918,#117919);
#101316=AXIS2_PLACEMENT_3D('',#183165,#117921,#117922);
#101317=AXIS2_PLACEMENT_3D('',#183169,#117925,#117926);
#101318=AXIS2_PLACEMENT_3D('',#183172,#117927,#117928);
#101319=AXIS2_PLACEMENT_3D('',#183180,#117932,#117933);
#101320=AXIS2_PLACEMENT_3D('',#183186,#117936,#117937);
#101321=AXIS2_PLACEMENT_3D('',#183190,#117939,#117940);
#101322=AXIS2_PLACEMENT_3D('',#183194,#117943,#117944);
#101323=AXIS2_PLACEMENT_3D('',#183199,#117946,#117947);
#101324=AXIS2_PLACEMENT_3D('',#183202,#117949,#117950);
#101325=AXIS2_PLACEMENT_3D('',#183203,#117951,#117952);
#101326=AXIS2_PLACEMENT_3D('',#183206,#117953,#117954);
#101327=AXIS2_PLACEMENT_3D('',#183214,#117958,#117959);
#101328=AXIS2_PLACEMENT_3D('',#183220,#117962,#117963);
#101329=AXIS2_PLACEMENT_3D('',#183224,#117965,#117966);
#101330=AXIS2_PLACEMENT_3D('',#183228,#117969,#117970);
#101331=AXIS2_PLACEMENT_3D('',#183231,#117971,#117972);
#101332=AXIS2_PLACEMENT_3D('',#183239,#117976,#117977);
#101333=AXIS2_PLACEMENT_3D('',#183245,#117980,#117981);
#101334=AXIS2_PLACEMENT_3D('',#183249,#117983,#117984);
#101335=AXIS2_PLACEMENT_3D('',#183253,#117987,#117988);
#101336=AXIS2_PLACEMENT_3D('',#183258,#117990,#117991);
#101337=AXIS2_PLACEMENT_3D('',#183261,#117993,#117994);
#101338=AXIS2_PLACEMENT_3D('',#183262,#117995,#117996);
#101339=AXIS2_PLACEMENT_3D('',#183265,#117997,#117998);
#101340=AXIS2_PLACEMENT_3D('',#183273,#118002,#118003);
#101341=AXIS2_PLACEMENT_3D('',#183279,#118006,#118007);
#101342=AXIS2_PLACEMENT_3D('',#183283,#118009,#118010);
#101343=AXIS2_PLACEMENT_3D('',#183287,#118013,#118014);
#101344=AXIS2_PLACEMENT_3D('',#183290,#118015,#118016);
#101345=AXIS2_PLACEMENT_3D('',#183298,#118020,#118021);
#101346=AXIS2_PLACEMENT_3D('',#183304,#118024,#118025);
#101347=AXIS2_PLACEMENT_3D('',#183308,#118027,#118028);
#101348=AXIS2_PLACEMENT_3D('',#183312,#118031,#118032);
#101349=AXIS2_PLACEMENT_3D('',#183317,#118034,#118035);
#101350=AXIS2_PLACEMENT_3D('',#183320,#118037,#118038);
#101351=AXIS2_PLACEMENT_3D('',#183321,#118039,#118040);
#101352=AXIS2_PLACEMENT_3D('',#183324,#118041,#118042);
#101353=AXIS2_PLACEMENT_3D('',#183332,#118046,#118047);
#101354=AXIS2_PLACEMENT_3D('',#183338,#118050,#118051);
#101355=AXIS2_PLACEMENT_3D('',#183342,#118053,#118054);
#101356=AXIS2_PLACEMENT_3D('',#183346,#118057,#118058);
#101357=AXIS2_PLACEMENT_3D('',#183349,#118059,#118060);
#101358=AXIS2_PLACEMENT_3D('',#183357,#118064,#118065);
#101359=AXIS2_PLACEMENT_3D('',#183363,#118068,#118069);
#101360=AXIS2_PLACEMENT_3D('',#183367,#118071,#118072);
#101361=AXIS2_PLACEMENT_3D('',#183371,#118075,#118076);
#101362=AXIS2_PLACEMENT_3D('',#183376,#118078,#118079);
#101363=AXIS2_PLACEMENT_3D('',#183379,#118081,#118082);
#101364=AXIS2_PLACEMENT_3D('',#183380,#118083,#118084);
#101365=AXIS2_PLACEMENT_3D('',#183383,#118085,#118086);
#101366=AXIS2_PLACEMENT_3D('',#183391,#118090,#118091);
#101367=AXIS2_PLACEMENT_3D('',#183397,#118094,#118095);
#101368=AXIS2_PLACEMENT_3D('',#183401,#118097,#118098);
#101369=AXIS2_PLACEMENT_3D('',#183405,#118101,#118102);
#101370=AXIS2_PLACEMENT_3D('',#183408,#118103,#118104);
#101371=AXIS2_PLACEMENT_3D('',#183416,#118108,#118109);
#101372=AXIS2_PLACEMENT_3D('',#183422,#118112,#118113);
#101373=AXIS2_PLACEMENT_3D('',#183426,#118115,#118116);
#101374=AXIS2_PLACEMENT_3D('',#183430,#118119,#118120);
#101375=AXIS2_PLACEMENT_3D('',#183435,#118122,#118123);
#101376=AXIS2_PLACEMENT_3D('',#183438,#118125,#118126);
#101377=AXIS2_PLACEMENT_3D('',#183439,#118127,#118128);
#101378=AXIS2_PLACEMENT_3D('',#183442,#118129,#118130);
#101379=AXIS2_PLACEMENT_3D('',#183450,#118134,#118135);
#101380=AXIS2_PLACEMENT_3D('',#183456,#118138,#118139);
#101381=AXIS2_PLACEMENT_3D('',#183460,#118141,#118142);
#101382=AXIS2_PLACEMENT_3D('',#183464,#118145,#118146);
#101383=AXIS2_PLACEMENT_3D('',#183467,#118147,#118148);
#101384=AXIS2_PLACEMENT_3D('',#183475,#118152,#118153);
#101385=AXIS2_PLACEMENT_3D('',#183481,#118156,#118157);
#101386=AXIS2_PLACEMENT_3D('',#183485,#118159,#118160);
#101387=AXIS2_PLACEMENT_3D('',#183489,#118163,#118164);
#101388=AXIS2_PLACEMENT_3D('',#183494,#118166,#118167);
#101389=AXIS2_PLACEMENT_3D('',#183497,#118169,#118170);
#101390=AXIS2_PLACEMENT_3D('',#183498,#118171,#118172);
#101391=AXIS2_PLACEMENT_3D('',#183501,#118173,#118174);
#101392=AXIS2_PLACEMENT_3D('',#183509,#118178,#118179);
#101393=AXIS2_PLACEMENT_3D('',#183515,#118182,#118183);
#101394=AXIS2_PLACEMENT_3D('',#183519,#118185,#118186);
#101395=AXIS2_PLACEMENT_3D('',#183523,#118189,#118190);
#101396=AXIS2_PLACEMENT_3D('',#183526,#118191,#118192);
#101397=AXIS2_PLACEMENT_3D('',#183534,#118196,#118197);
#101398=AXIS2_PLACEMENT_3D('',#183540,#118200,#118201);
#101399=AXIS2_PLACEMENT_3D('',#183544,#118203,#118204);
#101400=AXIS2_PLACEMENT_3D('',#183548,#118207,#118208);
#101401=AXIS2_PLACEMENT_3D('',#183553,#118210,#118211);
#101402=AXIS2_PLACEMENT_3D('',#183556,#118213,#118214);
#101403=AXIS2_PLACEMENT_3D('',#183557,#118215,#118216);
#101404=AXIS2_PLACEMENT_3D('',#183560,#118217,#118218);
#101405=AXIS2_PLACEMENT_3D('',#183568,#118222,#118223);
#101406=AXIS2_PLACEMENT_3D('',#183574,#118226,#118227);
#101407=AXIS2_PLACEMENT_3D('',#183578,#118229,#118230);
#101408=AXIS2_PLACEMENT_3D('',#183582,#118233,#118234);
#101409=AXIS2_PLACEMENT_3D('',#183585,#118235,#118236);
#101410=AXIS2_PLACEMENT_3D('',#183593,#118240,#118241);
#101411=AXIS2_PLACEMENT_3D('',#183599,#118244,#118245);
#101412=AXIS2_PLACEMENT_3D('',#183603,#118247,#118248);
#101413=AXIS2_PLACEMENT_3D('',#183607,#118251,#118252);
#101414=AXIS2_PLACEMENT_3D('',#183612,#118254,#118255);
#101415=AXIS2_PLACEMENT_3D('',#183615,#118257,#118258);
#101416=AXIS2_PLACEMENT_3D('',#183616,#118259,#118260);
#101417=AXIS2_PLACEMENT_3D('',#183619,#118261,#118262);
#101418=AXIS2_PLACEMENT_3D('',#183627,#118266,#118267);
#101419=AXIS2_PLACEMENT_3D('',#183633,#118270,#118271);
#101420=AXIS2_PLACEMENT_3D('',#183637,#118273,#118274);
#101421=AXIS2_PLACEMENT_3D('',#183641,#118277,#118278);
#101422=AXIS2_PLACEMENT_3D('',#183644,#118279,#118280);
#101423=AXIS2_PLACEMENT_3D('',#183652,#118284,#118285);
#101424=AXIS2_PLACEMENT_3D('',#183658,#118288,#118289);
#101425=AXIS2_PLACEMENT_3D('',#183662,#118291,#118292);
#101426=AXIS2_PLACEMENT_3D('',#183666,#118295,#118296);
#101427=AXIS2_PLACEMENT_3D('',#183671,#118298,#118299);
#101428=AXIS2_PLACEMENT_3D('',#183674,#118301,#118302);
#101429=AXIS2_PLACEMENT_3D('',#183675,#118303,#118304);
#101430=AXIS2_PLACEMENT_3D('',#183678,#118305,#118306);
#101431=AXIS2_PLACEMENT_3D('',#183686,#118310,#118311);
#101432=AXIS2_PLACEMENT_3D('',#183692,#118314,#118315);
#101433=AXIS2_PLACEMENT_3D('',#183696,#118317,#118318);
#101434=AXIS2_PLACEMENT_3D('',#183700,#118321,#118322);
#101435=AXIS2_PLACEMENT_3D('',#183703,#118323,#118324);
#101436=AXIS2_PLACEMENT_3D('',#183711,#118328,#118329);
#101437=AXIS2_PLACEMENT_3D('',#183717,#118332,#118333);
#101438=AXIS2_PLACEMENT_3D('',#183721,#118335,#118336);
#101439=AXIS2_PLACEMENT_3D('',#183725,#118339,#118340);
#101440=AXIS2_PLACEMENT_3D('',#183730,#118342,#118343);
#101441=AXIS2_PLACEMENT_3D('',#183733,#118345,#118346);
#101442=AXIS2_PLACEMENT_3D('',#183734,#118347,#118348);
#101443=AXIS2_PLACEMENT_3D('',#183737,#118349,#118350);
#101444=AXIS2_PLACEMENT_3D('',#183745,#118354,#118355);
#101445=AXIS2_PLACEMENT_3D('',#183751,#118358,#118359);
#101446=AXIS2_PLACEMENT_3D('',#183755,#118361,#118362);
#101447=AXIS2_PLACEMENT_3D('',#183759,#118365,#118366);
#101448=AXIS2_PLACEMENT_3D('',#183762,#118367,#118368);
#101449=AXIS2_PLACEMENT_3D('',#183770,#118372,#118373);
#101450=AXIS2_PLACEMENT_3D('',#183776,#118376,#118377);
#101451=AXIS2_PLACEMENT_3D('',#183780,#118379,#118380);
#101452=AXIS2_PLACEMENT_3D('',#183784,#118383,#118384);
#101453=AXIS2_PLACEMENT_3D('',#183789,#118386,#118387);
#101454=AXIS2_PLACEMENT_3D('',#183792,#118389,#118390);
#101455=AXIS2_PLACEMENT_3D('',#183793,#118391,#118392);
#101456=AXIS2_PLACEMENT_3D('',#183796,#118393,#118394);
#101457=AXIS2_PLACEMENT_3D('',#183804,#118398,#118399);
#101458=AXIS2_PLACEMENT_3D('',#183810,#118402,#118403);
#101459=AXIS2_PLACEMENT_3D('',#183814,#118405,#118406);
#101460=AXIS2_PLACEMENT_3D('',#183818,#118409,#118410);
#101461=AXIS2_PLACEMENT_3D('',#183821,#118411,#118412);
#101462=AXIS2_PLACEMENT_3D('',#183829,#118416,#118417);
#101463=AXIS2_PLACEMENT_3D('',#183835,#118420,#118421);
#101464=AXIS2_PLACEMENT_3D('',#183839,#118423,#118424);
#101465=AXIS2_PLACEMENT_3D('',#183843,#118427,#118428);
#101466=AXIS2_PLACEMENT_3D('',#183848,#118430,#118431);
#101467=AXIS2_PLACEMENT_3D('',#183851,#118433,#118434);
#101468=AXIS2_PLACEMENT_3D('',#183852,#118435,#118436);
#101469=AXIS2_PLACEMENT_3D('',#183855,#118437,#118438);
#101470=AXIS2_PLACEMENT_3D('',#183863,#118442,#118443);
#101471=AXIS2_PLACEMENT_3D('',#183869,#118446,#118447);
#101472=AXIS2_PLACEMENT_3D('',#183873,#118449,#118450);
#101473=AXIS2_PLACEMENT_3D('',#183877,#118453,#118454);
#101474=AXIS2_PLACEMENT_3D('',#183880,#118455,#118456);
#101475=AXIS2_PLACEMENT_3D('',#183888,#118460,#118461);
#101476=AXIS2_PLACEMENT_3D('',#183894,#118464,#118465);
#101477=AXIS2_PLACEMENT_3D('',#183898,#118467,#118468);
#101478=AXIS2_PLACEMENT_3D('',#183902,#118471,#118472);
#101479=AXIS2_PLACEMENT_3D('',#183907,#118474,#118475);
#101480=AXIS2_PLACEMENT_3D('',#183910,#118477,#118478);
#101481=AXIS2_PLACEMENT_3D('',#183911,#118479,#118480);
#101482=AXIS2_PLACEMENT_3D('',#183914,#118481,#118482);
#101483=AXIS2_PLACEMENT_3D('',#183922,#118486,#118487);
#101484=AXIS2_PLACEMENT_3D('',#183928,#118490,#118491);
#101485=AXIS2_PLACEMENT_3D('',#183932,#118493,#118494);
#101486=AXIS2_PLACEMENT_3D('',#183936,#118497,#118498);
#101487=AXIS2_PLACEMENT_3D('',#183939,#118499,#118500);
#101488=AXIS2_PLACEMENT_3D('',#183947,#118504,#118505);
#101489=AXIS2_PLACEMENT_3D('',#183953,#118508,#118509);
#101490=AXIS2_PLACEMENT_3D('',#183957,#118511,#118512);
#101491=AXIS2_PLACEMENT_3D('',#183961,#118515,#118516);
#101492=AXIS2_PLACEMENT_3D('',#183966,#118518,#118519);
#101493=AXIS2_PLACEMENT_3D('',#183969,#118521,#118522);
#101494=AXIS2_PLACEMENT_3D('',#183970,#118523,#118524);
#101495=AXIS2_PLACEMENT_3D('',#183973,#118525,#118526);
#101496=AXIS2_PLACEMENT_3D('',#183981,#118530,#118531);
#101497=AXIS2_PLACEMENT_3D('',#183987,#118534,#118535);
#101498=AXIS2_PLACEMENT_3D('',#183991,#118537,#118538);
#101499=AXIS2_PLACEMENT_3D('',#183995,#118541,#118542);
#101500=AXIS2_PLACEMENT_3D('',#183998,#118543,#118544);
#101501=AXIS2_PLACEMENT_3D('',#184006,#118548,#118549);
#101502=AXIS2_PLACEMENT_3D('',#184012,#118552,#118553);
#101503=AXIS2_PLACEMENT_3D('',#184016,#118555,#118556);
#101504=AXIS2_PLACEMENT_3D('',#184020,#118559,#118560);
#101505=AXIS2_PLACEMENT_3D('',#184025,#118562,#118563);
#101506=AXIS2_PLACEMENT_3D('',#184028,#118565,#118566);
#101507=AXIS2_PLACEMENT_3D('',#184029,#118567,#118568);
#101508=AXIS2_PLACEMENT_3D('',#184032,#118569,#118570);
#101509=AXIS2_PLACEMENT_3D('',#184040,#118574,#118575);
#101510=AXIS2_PLACEMENT_3D('',#184046,#118578,#118579);
#101511=AXIS2_PLACEMENT_3D('',#184050,#118581,#118582);
#101512=AXIS2_PLACEMENT_3D('',#184054,#118585,#118586);
#101513=AXIS2_PLACEMENT_3D('',#184057,#118587,#118588);
#101514=AXIS2_PLACEMENT_3D('',#184065,#118592,#118593);
#101515=AXIS2_PLACEMENT_3D('',#184071,#118596,#118597);
#101516=AXIS2_PLACEMENT_3D('',#184075,#118599,#118600);
#101517=AXIS2_PLACEMENT_3D('',#184079,#118603,#118604);
#101518=AXIS2_PLACEMENT_3D('',#184084,#118606,#118607);
#101519=AXIS2_PLACEMENT_3D('',#184087,#118609,#118610);
#101520=AXIS2_PLACEMENT_3D('',#184088,#118611,#118612);
#101521=AXIS2_PLACEMENT_3D('',#184091,#118613,#118614);
#101522=AXIS2_PLACEMENT_3D('',#184099,#118618,#118619);
#101523=AXIS2_PLACEMENT_3D('',#184105,#118622,#118623);
#101524=AXIS2_PLACEMENT_3D('',#184109,#118625,#118626);
#101525=AXIS2_PLACEMENT_3D('',#184113,#118629,#118630);
#101526=AXIS2_PLACEMENT_3D('',#184116,#118631,#118632);
#101527=AXIS2_PLACEMENT_3D('',#184124,#118636,#118637);
#101528=AXIS2_PLACEMENT_3D('',#184130,#118640,#118641);
#101529=AXIS2_PLACEMENT_3D('',#184134,#118643,#118644);
#101530=AXIS2_PLACEMENT_3D('',#184138,#118647,#118648);
#101531=AXIS2_PLACEMENT_3D('',#184143,#118650,#118651);
#101532=AXIS2_PLACEMENT_3D('',#184146,#118653,#118654);
#101533=AXIS2_PLACEMENT_3D('',#184147,#118655,#118656);
#101534=AXIS2_PLACEMENT_3D('',#184150,#118657,#118658);
#101535=AXIS2_PLACEMENT_3D('',#184158,#118662,#118663);
#101536=AXIS2_PLACEMENT_3D('',#184164,#118666,#118667);
#101537=AXIS2_PLACEMENT_3D('',#184168,#118669,#118670);
#101538=AXIS2_PLACEMENT_3D('',#184172,#118673,#118674);
#101539=AXIS2_PLACEMENT_3D('',#184175,#118675,#118676);
#101540=AXIS2_PLACEMENT_3D('',#184183,#118680,#118681);
#101541=AXIS2_PLACEMENT_3D('',#184189,#118684,#118685);
#101542=AXIS2_PLACEMENT_3D('',#184193,#118687,#118688);
#101543=AXIS2_PLACEMENT_3D('',#184197,#118691,#118692);
#101544=AXIS2_PLACEMENT_3D('',#184200,#118695,#118696);
#101545=AXIS2_PLACEMENT_3D('',#184203,#118697,#118698);
#101546=AXIS2_PLACEMENT_3D('',#184211,#118702,#118703);
#101547=AXIS2_PLACEMENT_3D('',#184217,#118706,#118707);
#101548=AXIS2_PLACEMENT_3D('',#184221,#118709,#118710);
#101549=AXIS2_PLACEMENT_3D('',#184225,#118713,#118714);
#101550=AXIS2_PLACEMENT_3D('',#184228,#118715,#118716);
#101551=AXIS2_PLACEMENT_3D('',#184236,#118720,#118721);
#101552=AXIS2_PLACEMENT_3D('',#184242,#118724,#118725);
#101553=AXIS2_PLACEMENT_3D('',#184246,#118727,#118728);
#101554=AXIS2_PLACEMENT_3D('',#184250,#118731,#118732);
#101555=AXIS2_PLACEMENT_3D('',#184255,#118734,#118735);
#101556=AXIS2_PLACEMENT_3D('',#184258,#118737,#118738);
#101557=AXIS2_PLACEMENT_3D('',#184259,#118739,#118740);
#101558=AXIS2_PLACEMENT_3D('',#184262,#118741,#118742);
#101559=AXIS2_PLACEMENT_3D('',#184270,#118746,#118747);
#101560=AXIS2_PLACEMENT_3D('',#184276,#118750,#118751);
#101561=AXIS2_PLACEMENT_3D('',#184280,#118753,#118754);
#101562=AXIS2_PLACEMENT_3D('',#184284,#118757,#118758);
#101563=AXIS2_PLACEMENT_3D('',#184287,#118759,#118760);
#101564=AXIS2_PLACEMENT_3D('',#184295,#118764,#118765);
#101565=AXIS2_PLACEMENT_3D('',#184301,#118768,#118769);
#101566=AXIS2_PLACEMENT_3D('',#184305,#118771,#118772);
#101567=AXIS2_PLACEMENT_3D('',#184309,#118775,#118776);
#101568=AXIS2_PLACEMENT_3D('',#184314,#118778,#118779);
#101569=AXIS2_PLACEMENT_3D('',#184317,#118781,#118782);
#101570=AXIS2_PLACEMENT_3D('',#184318,#118783,#118784);
#101571=AXIS2_PLACEMENT_3D('',#184321,#118785,#118786);
#101572=AXIS2_PLACEMENT_3D('',#184329,#118790,#118791);
#101573=AXIS2_PLACEMENT_3D('',#184335,#118794,#118795);
#101574=AXIS2_PLACEMENT_3D('',#184339,#118797,#118798);
#101575=AXIS2_PLACEMENT_3D('',#184343,#118801,#118802);
#101576=AXIS2_PLACEMENT_3D('',#184346,#118803,#118804);
#101577=AXIS2_PLACEMENT_3D('',#184354,#118808,#118809);
#101578=AXIS2_PLACEMENT_3D('',#184360,#118812,#118813);
#101579=AXIS2_PLACEMENT_3D('',#184364,#118815,#118816);
#101580=AXIS2_PLACEMENT_3D('',#184368,#118819,#118820);
#101581=AXIS2_PLACEMENT_3D('',#184373,#118822,#118823);
#101582=AXIS2_PLACEMENT_3D('',#184376,#118825,#118826);
#101583=AXIS2_PLACEMENT_3D('',#184377,#118827,#118828);
#101584=AXIS2_PLACEMENT_3D('',#184380,#118829,#118830);
#101585=AXIS2_PLACEMENT_3D('',#184388,#118834,#118835);
#101586=AXIS2_PLACEMENT_3D('',#184394,#118838,#118839);
#101587=AXIS2_PLACEMENT_3D('',#184398,#118841,#118842);
#101588=AXIS2_PLACEMENT_3D('',#184402,#118845,#118846);
#101589=AXIS2_PLACEMENT_3D('',#184405,#118847,#118848);
#101590=AXIS2_PLACEMENT_3D('',#184413,#118852,#118853);
#101591=AXIS2_PLACEMENT_3D('',#184419,#118856,#118857);
#101592=AXIS2_PLACEMENT_3D('',#184423,#118859,#118860);
#101593=AXIS2_PLACEMENT_3D('',#184427,#118863,#118864);
#101594=AXIS2_PLACEMENT_3D('',#184432,#118866,#118867);
#101595=AXIS2_PLACEMENT_3D('',#184435,#118869,#118870);
#101596=AXIS2_PLACEMENT_3D('',#184436,#118871,#118872);
#101597=AXIS2_PLACEMENT_3D('',#184439,#118873,#118874);
#101598=AXIS2_PLACEMENT_3D('',#184447,#118878,#118879);
#101599=AXIS2_PLACEMENT_3D('',#184453,#118882,#118883);
#101600=AXIS2_PLACEMENT_3D('',#184457,#118885,#118886);
#101601=AXIS2_PLACEMENT_3D('',#184461,#118889,#118890);
#101602=AXIS2_PLACEMENT_3D('',#184464,#118891,#118892);
#101603=AXIS2_PLACEMENT_3D('',#184472,#118896,#118897);
#101604=AXIS2_PLACEMENT_3D('',#184478,#118900,#118901);
#101605=AXIS2_PLACEMENT_3D('',#184482,#118903,#118904);
#101606=AXIS2_PLACEMENT_3D('',#184486,#118907,#118908);
#101607=AXIS2_PLACEMENT_3D('',#184491,#118910,#118911);
#101608=AXIS2_PLACEMENT_3D('',#184494,#118913,#118914);
#101609=AXIS2_PLACEMENT_3D('',#184495,#118915,#118916);
#101610=AXIS2_PLACEMENT_3D('',#184498,#118917,#118918);
#101611=AXIS2_PLACEMENT_3D('',#184506,#118922,#118923);
#101612=AXIS2_PLACEMENT_3D('',#184512,#118926,#118927);
#101613=AXIS2_PLACEMENT_3D('',#184516,#118929,#118930);
#101614=AXIS2_PLACEMENT_3D('',#184520,#118933,#118934);
#101615=AXIS2_PLACEMENT_3D('',#184523,#118935,#118936);
#101616=AXIS2_PLACEMENT_3D('',#184531,#118940,#118941);
#101617=AXIS2_PLACEMENT_3D('',#184537,#118944,#118945);
#101618=AXIS2_PLACEMENT_3D('',#184541,#118947,#118948);
#101619=AXIS2_PLACEMENT_3D('',#184545,#118951,#118952);
#101620=AXIS2_PLACEMENT_3D('',#184550,#118954,#118955);
#101621=AXIS2_PLACEMENT_3D('',#184553,#118957,#118958);
#101622=AXIS2_PLACEMENT_3D('',#184554,#118959,#118960);
#101623=AXIS2_PLACEMENT_3D('',#184557,#118961,#118962);
#101624=AXIS2_PLACEMENT_3D('',#184565,#118966,#118967);
#101625=AXIS2_PLACEMENT_3D('',#184571,#118970,#118971);
#101626=AXIS2_PLACEMENT_3D('',#184575,#118973,#118974);
#101627=AXIS2_PLACEMENT_3D('',#184579,#118977,#118978);
#101628=AXIS2_PLACEMENT_3D('',#184582,#118979,#118980);
#101629=AXIS2_PLACEMENT_3D('',#184590,#118984,#118985);
#101630=AXIS2_PLACEMENT_3D('',#184596,#118988,#118989);
#101631=AXIS2_PLACEMENT_3D('',#184600,#118991,#118992);
#101632=AXIS2_PLACEMENT_3D('',#184604,#118995,#118996);
#101633=AXIS2_PLACEMENT_3D('',#184609,#118998,#118999);
#101634=AXIS2_PLACEMENT_3D('',#184612,#119001,#119002);
#101635=AXIS2_PLACEMENT_3D('',#184613,#119003,#119004);
#101636=AXIS2_PLACEMENT_3D('',#184616,#119005,#119006);
#101637=AXIS2_PLACEMENT_3D('',#184624,#119010,#119011);
#101638=AXIS2_PLACEMENT_3D('',#184630,#119014,#119015);
#101639=AXIS2_PLACEMENT_3D('',#184634,#119017,#119018);
#101640=AXIS2_PLACEMENT_3D('',#184638,#119021,#119022);
#101641=AXIS2_PLACEMENT_3D('',#184641,#119023,#119024);
#101642=AXIS2_PLACEMENT_3D('',#184649,#119028,#119029);
#101643=AXIS2_PLACEMENT_3D('',#184655,#119032,#119033);
#101644=AXIS2_PLACEMENT_3D('',#184659,#119035,#119036);
#101645=AXIS2_PLACEMENT_3D('',#184663,#119039,#119040);
#101646=AXIS2_PLACEMENT_3D('',#184668,#119042,#119043);
#101647=AXIS2_PLACEMENT_3D('',#184671,#119045,#119046);
#101648=AXIS2_PLACEMENT_3D('',#184672,#119047,#119048);
#101649=AXIS2_PLACEMENT_3D('',#184675,#119049,#119050);
#101650=AXIS2_PLACEMENT_3D('',#184683,#119054,#119055);
#101651=AXIS2_PLACEMENT_3D('',#184689,#119058,#119059);
#101652=AXIS2_PLACEMENT_3D('',#184693,#119061,#119062);
#101653=AXIS2_PLACEMENT_3D('',#184697,#119065,#119066);
#101654=AXIS2_PLACEMENT_3D('',#184700,#119067,#119068);
#101655=AXIS2_PLACEMENT_3D('',#184708,#119072,#119073);
#101656=AXIS2_PLACEMENT_3D('',#184714,#119076,#119077);
#101657=AXIS2_PLACEMENT_3D('',#184718,#119079,#119080);
#101658=AXIS2_PLACEMENT_3D('',#184722,#119083,#119084);
#101659=AXIS2_PLACEMENT_3D('',#184727,#119086,#119087);
#101660=AXIS2_PLACEMENT_3D('',#184730,#119089,#119090);
#101661=AXIS2_PLACEMENT_3D('',#184731,#119091,#119092);
#101662=AXIS2_PLACEMENT_3D('',#184734,#119093,#119094);
#101663=AXIS2_PLACEMENT_3D('',#184742,#119098,#119099);
#101664=AXIS2_PLACEMENT_3D('',#184748,#119102,#119103);
#101665=AXIS2_PLACEMENT_3D('',#184752,#119105,#119106);
#101666=AXIS2_PLACEMENT_3D('',#184756,#119109,#119110);
#101667=AXIS2_PLACEMENT_3D('',#184759,#119111,#119112);
#101668=AXIS2_PLACEMENT_3D('',#184767,#119116,#119117);
#101669=AXIS2_PLACEMENT_3D('',#184773,#119120,#119121);
#101670=AXIS2_PLACEMENT_3D('',#184777,#119123,#119124);
#101671=AXIS2_PLACEMENT_3D('',#184781,#119127,#119128);
#101672=AXIS2_PLACEMENT_3D('',#184786,#119130,#119131);
#101673=AXIS2_PLACEMENT_3D('',#184789,#119133,#119134);
#101674=AXIS2_PLACEMENT_3D('',#184790,#119135,#119136);
#101675=AXIS2_PLACEMENT_3D('',#184793,#119137,#119138);
#101676=AXIS2_PLACEMENT_3D('',#184801,#119142,#119143);
#101677=AXIS2_PLACEMENT_3D('',#184807,#119146,#119147);
#101678=AXIS2_PLACEMENT_3D('',#184811,#119149,#119150);
#101679=AXIS2_PLACEMENT_3D('',#184815,#119153,#119154);
#101680=AXIS2_PLACEMENT_3D('',#184818,#119155,#119156);
#101681=AXIS2_PLACEMENT_3D('',#184826,#119160,#119161);
#101682=AXIS2_PLACEMENT_3D('',#184832,#119164,#119165);
#101683=AXIS2_PLACEMENT_3D('',#184836,#119167,#119168);
#101684=AXIS2_PLACEMENT_3D('',#184840,#119171,#119172);
#101685=AXIS2_PLACEMENT_3D('',#184845,#119174,#119175);
#101686=AXIS2_PLACEMENT_3D('',#184848,#119177,#119178);
#101687=AXIS2_PLACEMENT_3D('',#184849,#119179,#119180);
#101688=AXIS2_PLACEMENT_3D('',#184852,#119181,#119182);
#101689=AXIS2_PLACEMENT_3D('',#184860,#119186,#119187);
#101690=AXIS2_PLACEMENT_3D('',#184866,#119190,#119191);
#101691=AXIS2_PLACEMENT_3D('',#184870,#119193,#119194);
#101692=AXIS2_PLACEMENT_3D('',#184874,#119197,#119198);
#101693=AXIS2_PLACEMENT_3D('',#184877,#119199,#119200);
#101694=AXIS2_PLACEMENT_3D('',#184885,#119204,#119205);
#101695=AXIS2_PLACEMENT_3D('',#184891,#119208,#119209);
#101696=AXIS2_PLACEMENT_3D('',#184895,#119211,#119212);
#101697=AXIS2_PLACEMENT_3D('',#184899,#119215,#119216);
#101698=AXIS2_PLACEMENT_3D('',#184904,#119218,#119219);
#101699=AXIS2_PLACEMENT_3D('',#184907,#119221,#119222);
#101700=AXIS2_PLACEMENT_3D('',#184908,#119223,#119224);
#101701=AXIS2_PLACEMENT_3D('',#184911,#119225,#119226);
#101702=AXIS2_PLACEMENT_3D('',#184919,#119230,#119231);
#101703=AXIS2_PLACEMENT_3D('',#184925,#119234,#119235);
#101704=AXIS2_PLACEMENT_3D('',#184929,#119237,#119238);
#101705=AXIS2_PLACEMENT_3D('',#184933,#119241,#119242);
#101706=AXIS2_PLACEMENT_3D('',#184936,#119243,#119244);
#101707=AXIS2_PLACEMENT_3D('',#184944,#119248,#119249);
#101708=AXIS2_PLACEMENT_3D('',#184950,#119252,#119253);
#101709=AXIS2_PLACEMENT_3D('',#184954,#119255,#119256);
#101710=AXIS2_PLACEMENT_3D('',#184958,#119259,#119260);
#101711=AXIS2_PLACEMENT_3D('',#184963,#119262,#119263);
#101712=AXIS2_PLACEMENT_3D('',#184966,#119265,#119266);
#101713=AXIS2_PLACEMENT_3D('',#184967,#119267,#119268);
#101714=AXIS2_PLACEMENT_3D('',#184970,#119269,#119270);
#101715=AXIS2_PLACEMENT_3D('',#184978,#119274,#119275);
#101716=AXIS2_PLACEMENT_3D('',#184984,#119278,#119279);
#101717=AXIS2_PLACEMENT_3D('',#184988,#119281,#119282);
#101718=AXIS2_PLACEMENT_3D('',#184992,#119285,#119286);
#101719=AXIS2_PLACEMENT_3D('',#184995,#119287,#119288);
#101720=AXIS2_PLACEMENT_3D('',#185003,#119292,#119293);
#101721=AXIS2_PLACEMENT_3D('',#185009,#119296,#119297);
#101722=AXIS2_PLACEMENT_3D('',#185013,#119299,#119300);
#101723=AXIS2_PLACEMENT_3D('',#185017,#119303,#119304);
#101724=AXIS2_PLACEMENT_3D('',#185022,#119306,#119307);
#101725=AXIS2_PLACEMENT_3D('',#185025,#119309,#119310);
#101726=AXIS2_PLACEMENT_3D('',#185026,#119311,#119312);
#101727=AXIS2_PLACEMENT_3D('',#185029,#119313,#119314);
#101728=AXIS2_PLACEMENT_3D('',#185037,#119318,#119319);
#101729=AXIS2_PLACEMENT_3D('',#185043,#119322,#119323);
#101730=AXIS2_PLACEMENT_3D('',#185047,#119325,#119326);
#101731=AXIS2_PLACEMENT_3D('',#185051,#119329,#119330);
#101732=AXIS2_PLACEMENT_3D('',#185054,#119331,#119332);
#101733=AXIS2_PLACEMENT_3D('',#185062,#119336,#119337);
#101734=AXIS2_PLACEMENT_3D('',#185068,#119340,#119341);
#101735=AXIS2_PLACEMENT_3D('',#185072,#119343,#119344);
#101736=AXIS2_PLACEMENT_3D('',#185076,#119347,#119348);
#101737=AXIS2_PLACEMENT_3D('',#185079,#119351,#119352);
#101738=AXIS2_PLACEMENT_3D('',#185082,#119353,#119354);
#101739=AXIS2_PLACEMENT_3D('',#185090,#119358,#119359);
#101740=AXIS2_PLACEMENT_3D('',#185096,#119362,#119363);
#101741=AXIS2_PLACEMENT_3D('',#185100,#119365,#119366);
#101742=AXIS2_PLACEMENT_3D('',#185104,#119369,#119370);
#101743=AXIS2_PLACEMENT_3D('',#185107,#119371,#119372);
#101744=AXIS2_PLACEMENT_3D('',#185115,#119376,#119377);
#101745=AXIS2_PLACEMENT_3D('',#185121,#119380,#119381);
#101746=AXIS2_PLACEMENT_3D('',#185125,#119383,#119384);
#101747=AXIS2_PLACEMENT_3D('',#185129,#119387,#119388);
#101748=AXIS2_PLACEMENT_3D('',#185134,#119390,#119391);
#101749=AXIS2_PLACEMENT_3D('',#185137,#119393,#119394);
#101750=AXIS2_PLACEMENT_3D('',#185138,#119395,#119396);
#101751=AXIS2_PLACEMENT_3D('',#185141,#119397,#119398);
#101752=AXIS2_PLACEMENT_3D('',#185149,#119402,#119403);
#101753=AXIS2_PLACEMENT_3D('',#185155,#119406,#119407);
#101754=AXIS2_PLACEMENT_3D('',#185159,#119409,#119410);
#101755=AXIS2_PLACEMENT_3D('',#185163,#119413,#119414);
#101756=AXIS2_PLACEMENT_3D('',#185166,#119415,#119416);
#101757=AXIS2_PLACEMENT_3D('',#185174,#119420,#119421);
#101758=AXIS2_PLACEMENT_3D('',#185180,#119424,#119425);
#101759=AXIS2_PLACEMENT_3D('',#185184,#119427,#119428);
#101760=AXIS2_PLACEMENT_3D('',#185188,#119431,#119432);
#101761=AXIS2_PLACEMENT_3D('',#185193,#119434,#119435);
#101762=AXIS2_PLACEMENT_3D('',#185196,#119437,#119438);
#101763=AXIS2_PLACEMENT_3D('',#185197,#119439,#119440);
#101764=AXIS2_PLACEMENT_3D('',#185200,#119441,#119442);
#101765=AXIS2_PLACEMENT_3D('',#185208,#119446,#119447);
#101766=AXIS2_PLACEMENT_3D('',#185214,#119450,#119451);
#101767=AXIS2_PLACEMENT_3D('',#185218,#119453,#119454);
#101768=AXIS2_PLACEMENT_3D('',#185222,#119457,#119458);
#101769=AXIS2_PLACEMENT_3D('',#185225,#119459,#119460);
#101770=AXIS2_PLACEMENT_3D('',#185233,#119464,#119465);
#101771=AXIS2_PLACEMENT_3D('',#185239,#119468,#119469);
#101772=AXIS2_PLACEMENT_3D('',#185243,#119471,#119472);
#101773=AXIS2_PLACEMENT_3D('',#185247,#119475,#119476);
#101774=AXIS2_PLACEMENT_3D('',#185252,#119478,#119479);
#101775=AXIS2_PLACEMENT_3D('',#185255,#119481,#119482);
#101776=AXIS2_PLACEMENT_3D('',#185256,#119483,#119484);
#101777=AXIS2_PLACEMENT_3D('',#185259,#119485,#119486);
#101778=AXIS2_PLACEMENT_3D('',#185267,#119490,#119491);
#101779=AXIS2_PLACEMENT_3D('',#185273,#119494,#119495);
#101780=AXIS2_PLACEMENT_3D('',#185277,#119497,#119498);
#101781=AXIS2_PLACEMENT_3D('',#185281,#119501,#119502);
#101782=AXIS2_PLACEMENT_3D('',#185284,#119503,#119504);
#101783=AXIS2_PLACEMENT_3D('',#185292,#119508,#119509);
#101784=AXIS2_PLACEMENT_3D('',#185298,#119512,#119513);
#101785=AXIS2_PLACEMENT_3D('',#185302,#119515,#119516);
#101786=AXIS2_PLACEMENT_3D('',#185306,#119519,#119520);
#101787=AXIS2_PLACEMENT_3D('',#185311,#119522,#119523);
#101788=AXIS2_PLACEMENT_3D('',#185314,#119525,#119526);
#101789=AXIS2_PLACEMENT_3D('',#185315,#119527,#119528);
#101790=AXIS2_PLACEMENT_3D('',#185318,#119529,#119530);
#101791=AXIS2_PLACEMENT_3D('',#185326,#119534,#119535);
#101792=AXIS2_PLACEMENT_3D('',#185332,#119538,#119539);
#101793=AXIS2_PLACEMENT_3D('',#185336,#119541,#119542);
#101794=AXIS2_PLACEMENT_3D('',#185340,#119545,#119546);
#101795=AXIS2_PLACEMENT_3D('',#185343,#119547,#119548);
#101796=AXIS2_PLACEMENT_3D('',#185351,#119552,#119553);
#101797=AXIS2_PLACEMENT_3D('',#185357,#119556,#119557);
#101798=AXIS2_PLACEMENT_3D('',#185361,#119559,#119560);
#101799=AXIS2_PLACEMENT_3D('',#185365,#119563,#119564);
#101800=AXIS2_PLACEMENT_3D('',#185370,#119566,#119567);
#101801=AXIS2_PLACEMENT_3D('',#185373,#119569,#119570);
#101802=AXIS2_PLACEMENT_3D('',#185374,#119571,#119572);
#101803=AXIS2_PLACEMENT_3D('',#185377,#119573,#119574);
#101804=AXIS2_PLACEMENT_3D('',#185385,#119578,#119579);
#101805=AXIS2_PLACEMENT_3D('',#185391,#119582,#119583);
#101806=AXIS2_PLACEMENT_3D('',#185395,#119585,#119586);
#101807=AXIS2_PLACEMENT_3D('',#185399,#119589,#119590);
#101808=AXIS2_PLACEMENT_3D('',#185402,#119591,#119592);
#101809=AXIS2_PLACEMENT_3D('',#185410,#119596,#119597);
#101810=AXIS2_PLACEMENT_3D('',#185416,#119600,#119601);
#101811=AXIS2_PLACEMENT_3D('',#185420,#119603,#119604);
#101812=AXIS2_PLACEMENT_3D('',#185424,#119607,#119608);
#101813=AXIS2_PLACEMENT_3D('',#185429,#119610,#119611);
#101814=AXIS2_PLACEMENT_3D('',#185432,#119613,#119614);
#101815=AXIS2_PLACEMENT_3D('',#185433,#119615,#119616);
#101816=AXIS2_PLACEMENT_3D('',#185436,#119617,#119618);
#101817=AXIS2_PLACEMENT_3D('',#185444,#119622,#119623);
#101818=AXIS2_PLACEMENT_3D('',#185450,#119626,#119627);
#101819=AXIS2_PLACEMENT_3D('',#185454,#119629,#119630);
#101820=AXIS2_PLACEMENT_3D('',#185458,#119633,#119634);
#101821=AXIS2_PLACEMENT_3D('',#185461,#119635,#119636);
#101822=AXIS2_PLACEMENT_3D('',#185469,#119640,#119641);
#101823=AXIS2_PLACEMENT_3D('',#185475,#119644,#119645);
#101824=AXIS2_PLACEMENT_3D('',#185479,#119647,#119648);
#101825=AXIS2_PLACEMENT_3D('',#185483,#119651,#119652);
#101826=AXIS2_PLACEMENT_3D('',#185488,#119654,#119655);
#101827=AXIS2_PLACEMENT_3D('',#185491,#119657,#119658);
#101828=AXIS2_PLACEMENT_3D('',#185492,#119659,#119660);
#101829=AXIS2_PLACEMENT_3D('',#185495,#119661,#119662);
#101830=AXIS2_PLACEMENT_3D('',#185503,#119666,#119667);
#101831=AXIS2_PLACEMENT_3D('',#185509,#119670,#119671);
#101832=AXIS2_PLACEMENT_3D('',#185513,#119673,#119674);
#101833=AXIS2_PLACEMENT_3D('',#185517,#119677,#119678);
#101834=AXIS2_PLACEMENT_3D('',#185520,#119679,#119680);
#101835=AXIS2_PLACEMENT_3D('',#185528,#119684,#119685);
#101836=AXIS2_PLACEMENT_3D('',#185534,#119688,#119689);
#101837=AXIS2_PLACEMENT_3D('',#185538,#119691,#119692);
#101838=AXIS2_PLACEMENT_3D('',#185542,#119695,#119696);
#101839=AXIS2_PLACEMENT_3D('',#185547,#119698,#119699);
#101840=AXIS2_PLACEMENT_3D('',#185550,#119701,#119702);
#101841=AXIS2_PLACEMENT_3D('',#185551,#119703,#119704);
#101842=AXIS2_PLACEMENT_3D('',#185554,#119705,#119706);
#101843=AXIS2_PLACEMENT_3D('',#185562,#119710,#119711);
#101844=AXIS2_PLACEMENT_3D('',#185568,#119714,#119715);
#101845=AXIS2_PLACEMENT_3D('',#185572,#119717,#119718);
#101846=AXIS2_PLACEMENT_3D('',#185576,#119721,#119722);
#101847=AXIS2_PLACEMENT_3D('',#185579,#119723,#119724);
#101848=AXIS2_PLACEMENT_3D('',#185587,#119728,#119729);
#101849=AXIS2_PLACEMENT_3D('',#185593,#119732,#119733);
#101850=AXIS2_PLACEMENT_3D('',#185597,#119735,#119736);
#101851=AXIS2_PLACEMENT_3D('',#185601,#119739,#119740);
#101852=AXIS2_PLACEMENT_3D('',#185606,#119742,#119743);
#101853=AXIS2_PLACEMENT_3D('',#185609,#119745,#119746);
#101854=AXIS2_PLACEMENT_3D('',#185610,#119747,#119748);
#101855=AXIS2_PLACEMENT_3D('',#185613,#119749,#119750);
#101856=AXIS2_PLACEMENT_3D('',#185621,#119754,#119755);
#101857=AXIS2_PLACEMENT_3D('',#185627,#119758,#119759);
#101858=AXIS2_PLACEMENT_3D('',#185631,#119761,#119762);
#101859=AXIS2_PLACEMENT_3D('',#185635,#119765,#119766);
#101860=AXIS2_PLACEMENT_3D('',#185638,#119767,#119768);
#101861=AXIS2_PLACEMENT_3D('',#185646,#119772,#119773);
#101862=AXIS2_PLACEMENT_3D('',#185652,#119776,#119777);
#101863=AXIS2_PLACEMENT_3D('',#185656,#119779,#119780);
#101864=AXIS2_PLACEMENT_3D('',#185660,#119783,#119784);
#101865=AXIS2_PLACEMENT_3D('',#185665,#119786,#119787);
#101866=AXIS2_PLACEMENT_3D('',#185668,#119789,#119790);
#101867=AXIS2_PLACEMENT_3D('',#185669,#119791,#119792);
#101868=AXIS2_PLACEMENT_3D('',#185672,#119793,#119794);
#101869=AXIS2_PLACEMENT_3D('',#185680,#119798,#119799);
#101870=AXIS2_PLACEMENT_3D('',#185686,#119802,#119803);
#101871=AXIS2_PLACEMENT_3D('',#185690,#119805,#119806);
#101872=AXIS2_PLACEMENT_3D('',#185694,#119809,#119810);
#101873=AXIS2_PLACEMENT_3D('',#185697,#119811,#119812);
#101874=AXIS2_PLACEMENT_3D('',#185705,#119816,#119817);
#101875=AXIS2_PLACEMENT_3D('',#185711,#119820,#119821);
#101876=AXIS2_PLACEMENT_3D('',#185715,#119823,#119824);
#101877=AXIS2_PLACEMENT_3D('',#185719,#119827,#119828);
#101878=AXIS2_PLACEMENT_3D('',#185724,#119830,#119831);
#101879=AXIS2_PLACEMENT_3D('',#185727,#119833,#119834);
#101880=AXIS2_PLACEMENT_3D('',#185728,#119835,#119836);
#101881=AXIS2_PLACEMENT_3D('',#185731,#119837,#119838);
#101882=AXIS2_PLACEMENT_3D('',#185739,#119842,#119843);
#101883=AXIS2_PLACEMENT_3D('',#185745,#119846,#119847);
#101884=AXIS2_PLACEMENT_3D('',#185749,#119849,#119850);
#101885=AXIS2_PLACEMENT_3D('',#185753,#119853,#119854);
#101886=AXIS2_PLACEMENT_3D('',#185756,#119855,#119856);
#101887=AXIS2_PLACEMENT_3D('',#185764,#119860,#119861);
#101888=AXIS2_PLACEMENT_3D('',#185770,#119864,#119865);
#101889=AXIS2_PLACEMENT_3D('',#185774,#119867,#119868);
#101890=AXIS2_PLACEMENT_3D('',#185778,#119871,#119872);
#101891=AXIS2_PLACEMENT_3D('',#185783,#119874,#119875);
#101892=AXIS2_PLACEMENT_3D('',#185786,#119877,#119878);
#101893=AXIS2_PLACEMENT_3D('',#185787,#119879,#119880);
#101894=AXIS2_PLACEMENT_3D('',#185790,#119881,#119882);
#101895=AXIS2_PLACEMENT_3D('',#185798,#119886,#119887);
#101896=AXIS2_PLACEMENT_3D('',#185804,#119890,#119891);
#101897=AXIS2_PLACEMENT_3D('',#185808,#119893,#119894);
#101898=AXIS2_PLACEMENT_3D('',#185812,#119897,#119898);
#101899=AXIS2_PLACEMENT_3D('',#185815,#119899,#119900);
#101900=AXIS2_PLACEMENT_3D('',#185823,#119904,#119905);
#101901=AXIS2_PLACEMENT_3D('',#185829,#119908,#119909);
#101902=AXIS2_PLACEMENT_3D('',#185833,#119911,#119912);
#101903=AXIS2_PLACEMENT_3D('',#185837,#119915,#119916);
#101904=AXIS2_PLACEMENT_3D('',#185842,#119918,#119919);
#101905=AXIS2_PLACEMENT_3D('',#185845,#119921,#119922);
#101906=AXIS2_PLACEMENT_3D('',#185846,#119923,#119924);
#101907=AXIS2_PLACEMENT_3D('',#185849,#119925,#119926);
#101908=AXIS2_PLACEMENT_3D('',#185857,#119930,#119931);
#101909=AXIS2_PLACEMENT_3D('',#185863,#119934,#119935);
#101910=AXIS2_PLACEMENT_3D('',#185867,#119937,#119938);
#101911=AXIS2_PLACEMENT_3D('',#185871,#119941,#119942);
#101912=AXIS2_PLACEMENT_3D('',#185874,#119943,#119944);
#101913=AXIS2_PLACEMENT_3D('',#185882,#119948,#119949);
#101914=AXIS2_PLACEMENT_3D('',#185888,#119952,#119953);
#101915=AXIS2_PLACEMENT_3D('',#185892,#119955,#119956);
#101916=AXIS2_PLACEMENT_3D('',#185896,#119959,#119960);
#101917=AXIS2_PLACEMENT_3D('',#185901,#119962,#119963);
#101918=AXIS2_PLACEMENT_3D('',#185904,#119965,#119966);
#101919=AXIS2_PLACEMENT_3D('',#185905,#119967,#119968);
#101920=AXIS2_PLACEMENT_3D('',#185908,#119969,#119970);
#101921=AXIS2_PLACEMENT_3D('',#185916,#119974,#119975);
#101922=AXIS2_PLACEMENT_3D('',#185922,#119978,#119979);
#101923=AXIS2_PLACEMENT_3D('',#185926,#119981,#119982);
#101924=AXIS2_PLACEMENT_3D('',#185930,#119985,#119986);
#101925=AXIS2_PLACEMENT_3D('',#185933,#119987,#119988);
#101926=AXIS2_PLACEMENT_3D('',#185941,#119992,#119993);
#101927=AXIS2_PLACEMENT_3D('',#185947,#119996,#119997);
#101928=AXIS2_PLACEMENT_3D('',#185951,#119999,#120000);
#101929=AXIS2_PLACEMENT_3D('',#185955,#120003,#120004);
#101930=AXIS2_PLACEMENT_3D('',#186060,#120005,#120006);
#101931=AXIS2_PLACEMENT_3D('',#186159,#120007,#120008);
#101932=AXIS2_PLACEMENT_3D('',#186264,#120009,#120010);
#101933=AXIS2_PLACEMENT_3D('',#186363,#120011,#120012);
#101934=AXIS2_PLACEMENT_3D('',#186468,#120013,#120014);
#101935=AXIS2_PLACEMENT_3D('',#186567,#120015,#120016);
#101936=AXIS2_PLACEMENT_3D('',#186672,#120017,#120018);
#101937=AXIS2_PLACEMENT_3D('',#186771,#120019,#120020);
#101938=AXIS2_PLACEMENT_3D('',#186876,#120021,#120022);
#101939=AXIS2_PLACEMENT_3D('',#186975,#120023,#120024);
#101940=AXIS2_PLACEMENT_3D('',#187080,#120025,#120026);
#101941=AXIS2_PLACEMENT_3D('',#187179,#120027,#120028);
#101942=AXIS2_PLACEMENT_3D('',#187284,#120029,#120030);
#101943=AXIS2_PLACEMENT_3D('',#187383,#120031,#120032);
#101944=AXIS2_PLACEMENT_3D('',#187488,#120033,#120034);
#101945=AXIS2_PLACEMENT_3D('',#187587,#120035,#120036);
#101946=AXIS2_PLACEMENT_3D('',#187692,#120037,#120038);
#101947=AXIS2_PLACEMENT_3D('',#187791,#120039,#120040);
#101948=AXIS2_PLACEMENT_3D('',#187896,#120041,#120042);
#101949=AXIS2_PLACEMENT_3D('',#187995,#120043,#120044);
#101950=AXIS2_PLACEMENT_3D('',#188100,#120045,#120046);
#101951=AXIS2_PLACEMENT_3D('',#188199,#120047,#120048);
#101952=AXIS2_PLACEMENT_3D('',#188304,#120049,#120050);
#101953=AXIS2_PLACEMENT_3D('',#188403,#120051,#120052);
#101954=AXIS2_PLACEMENT_3D('',#188508,#120053,#120054);
#101955=AXIS2_PLACEMENT_3D('',#188607,#120055,#120056);
#101956=AXIS2_PLACEMENT_3D('',#188712,#120057,#120058);
#101957=AXIS2_PLACEMENT_3D('',#188811,#120059,#120060);
#101958=AXIS2_PLACEMENT_3D('',#188916,#120061,#120062);
#101959=AXIS2_PLACEMENT_3D('',#189015,#120063,#120064);
#101960=AXIS2_PLACEMENT_3D('',#189120,#120065,#120066);
#101961=AXIS2_PLACEMENT_3D('',#189219,#120067,#120068);
#101962=AXIS2_PLACEMENT_3D('',#189324,#120069,#120070);
#101963=AXIS2_PLACEMENT_3D('',#189423,#120071,#120072);
#101964=AXIS2_PLACEMENT_3D('',#189528,#120073,#120074);
#101965=AXIS2_PLACEMENT_3D('',#189627,#120075,#120076);
#101966=AXIS2_PLACEMENT_3D('',#189732,#120077,#120078);
#101967=AXIS2_PLACEMENT_3D('',#189831,#120079,#120080);
#101968=AXIS2_PLACEMENT_3D('',#189936,#120081,#120082);
#101969=AXIS2_PLACEMENT_3D('',#190035,#120083,#120084);
#101970=AXIS2_PLACEMENT_3D('',#190140,#120085,#120086);
#101971=AXIS2_PLACEMENT_3D('',#190239,#120087,#120088);
#101972=AXIS2_PLACEMENT_3D('',#190344,#120089,#120090);
#101973=AXIS2_PLACEMENT_3D('',#190443,#120091,#120092);
#101974=AXIS2_PLACEMENT_3D('',#190548,#120093,#120094);
#101975=AXIS2_PLACEMENT_3D('',#190647,#120095,#120096);
#101976=AXIS2_PLACEMENT_3D('',#190752,#120097,#120098);
#101977=AXIS2_PLACEMENT_3D('',#190851,#120099,#120100);
#101978=AXIS2_PLACEMENT_3D('',#190956,#120101,#120102);
#101979=AXIS2_PLACEMENT_3D('',#191055,#120103,#120104);
#101980=AXIS2_PLACEMENT_3D('',#191160,#120105,#120106);
#101981=AXIS2_PLACEMENT_3D('',#191259,#120107,#120108);
#101982=AXIS2_PLACEMENT_3D('',#191364,#120109,#120110);
#101983=AXIS2_PLACEMENT_3D('',#191463,#120111,#120112);
#101984=AXIS2_PLACEMENT_3D('',#191568,#120113,#120114);
#101985=AXIS2_PLACEMENT_3D('',#191667,#120115,#120116);
#101986=AXIS2_PLACEMENT_3D('',#191772,#120117,#120118);
#101987=AXIS2_PLACEMENT_3D('',#191871,#120119,#120120);
#101988=AXIS2_PLACEMENT_3D('',#191976,#120121,#120122);
#101989=AXIS2_PLACEMENT_3D('',#192075,#120123,#120124);
#101990=AXIS2_PLACEMENT_3D('',#192180,#120125,#120126);
#101991=AXIS2_PLACEMENT_3D('',#192279,#120127,#120128);
#101992=AXIS2_PLACEMENT_3D('',#192384,#120129,#120130);
#101993=AXIS2_PLACEMENT_3D('',#192483,#120131,#120132);
#101994=AXIS2_PLACEMENT_3D('',#192588,#120133,#120134);
#101995=AXIS2_PLACEMENT_3D('',#192687,#120135,#120136);
#101996=AXIS2_PLACEMENT_3D('',#192792,#120137,#120138);
#101997=AXIS2_PLACEMENT_3D('',#192891,#120139,#120140);
#101998=AXIS2_PLACEMENT_3D('',#192996,#120141,#120142);
#101999=AXIS2_PLACEMENT_3D('',#193095,#120143,#120144);
#102000=AXIS2_PLACEMENT_3D('',#193200,#120145,#120146);
#102001=AXIS2_PLACEMENT_3D('',#193299,#120147,#120148);
#102002=AXIS2_PLACEMENT_3D('',#193404,#120149,#120150);
#102003=AXIS2_PLACEMENT_3D('',#193503,#120151,#120152);
#102004=AXIS2_PLACEMENT_3D('',#193608,#120153,#120154);
#102005=AXIS2_PLACEMENT_3D('',#193707,#120155,#120156);
#102006=AXIS2_PLACEMENT_3D('',#193812,#120157,#120158);
#102007=AXIS2_PLACEMENT_3D('',#193911,#120159,#120160);
#102008=AXIS2_PLACEMENT_3D('',#194016,#120161,#120162);
#102009=AXIS2_PLACEMENT_3D('',#194115,#120163,#120164);
#102010=AXIS2_PLACEMENT_3D('',#194220,#120165,#120166);
#102011=AXIS2_PLACEMENT_3D('',#194319,#120167,#120168);
#102012=AXIS2_PLACEMENT_3D('',#194424,#120169,#120170);
#102013=AXIS2_PLACEMENT_3D('',#194523,#120171,#120172);
#102014=AXIS2_PLACEMENT_3D('',#194628,#120173,#120174);
#102015=AXIS2_PLACEMENT_3D('',#194727,#120175,#120176);
#102016=AXIS2_PLACEMENT_3D('',#194832,#120177,#120178);
#102017=AXIS2_PLACEMENT_3D('',#194931,#120179,#120180);
#102018=AXIS2_PLACEMENT_3D('',#195036,#120181,#120182);
#102019=AXIS2_PLACEMENT_3D('',#195135,#120183,#120184);
#102020=AXIS2_PLACEMENT_3D('',#195240,#120185,#120186);
#102021=AXIS2_PLACEMENT_3D('',#195339,#120187,#120188);
#102022=AXIS2_PLACEMENT_3D('',#195444,#120189,#120190);
#102023=AXIS2_PLACEMENT_3D('',#195543,#120191,#120192);
#102024=AXIS2_PLACEMENT_3D('',#195648,#120193,#120194);
#102025=AXIS2_PLACEMENT_3D('',#195747,#120195,#120196);
#102026=AXIS2_PLACEMENT_3D('',#195852,#120197,#120198);
#102027=AXIS2_PLACEMENT_3D('',#195951,#120199,#120200);
#102028=AXIS2_PLACEMENT_3D('',#196056,#120201,#120202);
#102029=AXIS2_PLACEMENT_3D('',#196155,#120203,#120204);
#102030=AXIS2_PLACEMENT_3D('',#196260,#120205,#120206);
#102031=AXIS2_PLACEMENT_3D('',#196359,#120207,#120208);
#102032=AXIS2_PLACEMENT_3D('',#196464,#120209,#120210);
#102033=AXIS2_PLACEMENT_3D('',#196563,#120211,#120212);
#102034=AXIS2_PLACEMENT_3D('',#196668,#120213,#120214);
#102035=AXIS2_PLACEMENT_3D('',#196767,#120215,#120216);
#102036=AXIS2_PLACEMENT_3D('',#196872,#120217,#120218);
#102037=AXIS2_PLACEMENT_3D('',#196971,#120219,#120220);
#102038=AXIS2_PLACEMENT_3D('',#197076,#120221,#120222);
#102039=AXIS2_PLACEMENT_3D('',#197175,#120223,#120224);
#102040=AXIS2_PLACEMENT_3D('',#197280,#120225,#120226);
#102041=AXIS2_PLACEMENT_3D('',#197379,#120227,#120228);
#102042=AXIS2_PLACEMENT_3D('',#197484,#120229,#120230);
#102043=AXIS2_PLACEMENT_3D('',#197583,#120231,#120232);
#102044=AXIS2_PLACEMENT_3D('',#197688,#120233,#120234);
#102045=AXIS2_PLACEMENT_3D('',#197787,#120235,#120236);
#102046=AXIS2_PLACEMENT_3D('',#197892,#120237,#120238);
#102047=AXIS2_PLACEMENT_3D('',#197991,#120239,#120240);
#102048=AXIS2_PLACEMENT_3D('',#197992,#120241,#120242);
#102049=AXIS2_PLACEMENT_3D('',#197993,#120243,#120244);
#102050=AXIS2_PLACEMENT_3D('',#198006,#120245,#120246);
#102051=AXIS2_PLACEMENT_3D('',#198007,#120247,#120248);
#102052=AXIS2_PLACEMENT_3D('',#198008,#120249,#120250);
#102053=AXIS2_PLACEMENT_3D('',#198009,#120251,#120252);
#102054=AXIS2_PLACEMENT_3D('',#198010,#120253,#120254);
#102055=AXIS2_PLACEMENT_3D('',#198023,#120255,#120256);
#102056=AXIS2_PLACEMENT_3D('',#198036,#120257,#120258);
#102057=AXIS2_PLACEMENT_3D('',#198037,#120259,#120260);
#102058=AXIS2_PLACEMENT_3D('',#198038,#120261,#120262);
#102059=AXIS2_PLACEMENT_3D('',#198039,#120263,#120264);
#102060=AXIS2_PLACEMENT_3D('',#198040,#120265,#120266);
#102061=AXIS2_PLACEMENT_3D('',#198059,#120267,#120268);
#102062=AXIS2_PLACEMENT_3D('',#198060,#120269,#120270);
#102063=AXIS2_PLACEMENT_3D('',#198061,#120271,#120272);
#102064=AXIS2_PLACEMENT_3D('',#198062,#120273,#120274);
#102065=AXIS2_PLACEMENT_3D('',#198063,#120275,#120276);
#102066=AXIS2_PLACEMENT_3D('',#198076,#120277,#120278);
#102067=AXIS2_PLACEMENT_3D('',#198095,#120279,#120280);
#102068=AXIS2_PLACEMENT_3D('',#198096,#120281,#120282);
#102069=AXIS2_PLACEMENT_3D('',#198097,#120283,#120284);
#102070=AXIS2_PLACEMENT_3D('',#198098,#120285,#120286);
#102071=AXIS2_PLACEMENT_3D('',#198099,#120287,#120288);
#102072=AXIS2_PLACEMENT_3D('',#198118,#120289,#120290);
#102073=AXIS2_PLACEMENT_3D('',#198131,#120291,#120292);
#102074=AXIS2_PLACEMENT_3D('',#198132,#120293,#120294);
#102075=AXIS2_PLACEMENT_3D('',#198133,#120295,#120296);
#102076=AXIS2_PLACEMENT_3D('',#198134,#120297,#120298);
#102077=AXIS2_PLACEMENT_3D('',#198135,#120299,#120300);
#102078=AXIS2_PLACEMENT_3D('',#198154,#120301,#120302);
#102079=AXIS2_PLACEMENT_3D('',#198155,#120303,#120304);
#102080=AXIS2_PLACEMENT_3D('',#198156,#120305,#120306);
#102081=AXIS2_PLACEMENT_3D('',#198157,#120307,#120308);
#102082=AXIS2_PLACEMENT_3D('',#198158,#120309,#120310);
#102083=AXIS2_PLACEMENT_3D('',#198171,#120311,#120312);
#102084=AXIS2_PLACEMENT_3D('',#198184,#120313,#120314);
#102085=AXIS2_PLACEMENT_3D('',#198185,#120315,#120316);
#102086=AXIS2_PLACEMENT_3D('',#198186,#120317,#120318);
#102087=AXIS2_PLACEMENT_3D('',#198187,#120319,#120320);
#102088=AXIS2_PLACEMENT_3D('',#198188,#120321,#120322);
#102089=AXIS2_PLACEMENT_3D('',#198201,#120323,#120324);
#102090=AXIS2_PLACEMENT_3D('',#198202,#120325,#120326);
#102091=AXIS2_PLACEMENT_3D('',#198203,#120327,#120328);
#102092=AXIS2_PLACEMENT_3D('',#198204,#120329,#120330);
#102093=AXIS2_PLACEMENT_3D('',#198205,#120331,#120332);
#102094=AXIS2_PLACEMENT_3D('',#198218,#120333,#120334);
#102095=AXIS2_PLACEMENT_3D('',#198219,#120335,#120336);
#102096=AXIS2_PLACEMENT_3D('',#198220,#120337,#120338);
#102097=AXIS2_PLACEMENT_3D('',#198221,#120339,#120340);
#102098=AXIS2_PLACEMENT_3D('',#198222,#120341,#120342);
#102099=AXIS2_PLACEMENT_3D('',#198235,#120343,#120344);
#102100=AXIS2_PLACEMENT_3D('',#198248,#120345,#120346);
#102101=AXIS2_PLACEMENT_3D('',#198249,#120347,#120348);
#102102=AXIS2_PLACEMENT_3D('',#198250,#120349,#120350);
#102103=AXIS2_PLACEMENT_3D('',#198251,#120351,#120352);
#102104=AXIS2_PLACEMENT_3D('',#198252,#120353,#120354);
#102105=AXIS2_PLACEMENT_3D('',#198271,#120355,#120356);
#102106=AXIS2_PLACEMENT_3D('',#198272,#120357,#120358);
#102107=AXIS2_PLACEMENT_3D('',#198273,#120359,#120360);
#102108=AXIS2_PLACEMENT_3D('',#198274,#120361,#120362);
#102109=AXIS2_PLACEMENT_3D('',#198275,#120363,#120364);
#102110=AXIS2_PLACEMENT_3D('',#198288,#120365,#120366);
#102111=AXIS2_PLACEMENT_3D('',#198307,#120367,#120368);
#102112=AXIS2_PLACEMENT_3D('',#198308,#120369,#120370);
#102113=AXIS2_PLACEMENT_3D('',#198309,#120371,#120372);
#102114=AXIS2_PLACEMENT_3D('',#198310,#120373,#120374);
#102115=AXIS2_PLACEMENT_3D('',#198311,#120375,#120376);
#102116=AXIS2_PLACEMENT_3D('',#198330,#120377,#120378);
#102117=AXIS2_PLACEMENT_3D('',#198343,#120379,#120380);
#102118=AXIS2_PLACEMENT_3D('',#198344,#120381,#120382);
#102119=AXIS2_PLACEMENT_3D('',#198345,#120383,#120384);
#102120=AXIS2_PLACEMENT_3D('',#198346,#120385,#120386);
#102121=AXIS2_PLACEMENT_3D('',#198347,#120387,#120388);
#102122=AXIS2_PLACEMENT_3D('',#198366,#120389,#120390);
#102123=AXIS2_PLACEMENT_3D('',#198367,#120391,#120392);
#102124=AXIS2_PLACEMENT_3D('',#198368,#120393,#120394);
#102125=AXIS2_PLACEMENT_3D('',#198369,#120395,#120396);
#102126=AXIS2_PLACEMENT_3D('',#198370,#120397,#120398);
#102127=AXIS2_PLACEMENT_3D('',#198383,#120399,#120400);
#102128=AXIS2_PLACEMENT_3D('',#198396,#120401,#120402);
#102129=AXIS2_PLACEMENT_3D('',#198397,#120403,#120404);
#102130=AXIS2_PLACEMENT_3D('',#198398,#120405,#120406);
#102131=AXIS2_PLACEMENT_3D('',#198399,#120407,#120408);
#102132=AXIS2_PLACEMENT_3D('',#198400,#120409,#120410);
#102133=AXIS2_PLACEMENT_3D('',#198413,#120411,#120412);
#102134=AXIS2_PLACEMENT_3D('',#198414,#120413,#120414);
#102135=AXIS2_PLACEMENT_3D('',#198415,#120415,#120416);
#102136=AXIS2_PLACEMENT_3D('',#198416,#120417,#120418);
#102137=AXIS2_PLACEMENT_3D('',#198417,#120419,#120420);
#102138=AXIS2_PLACEMENT_3D('',#198430,#120421,#120422);
#102139=AXIS2_PLACEMENT_3D('',#198431,#120423,#120424);
#102140=AXIS2_PLACEMENT_3D('',#198432,#120425,#120426);
#102141=AXIS2_PLACEMENT_3D('',#198433,#120427,#120428);
#102142=AXIS2_PLACEMENT_3D('',#198434,#120429,#120430);
#102143=AXIS2_PLACEMENT_3D('',#198447,#120431,#120432);
#102144=AXIS2_PLACEMENT_3D('',#198460,#120433,#120434);
#102145=AXIS2_PLACEMENT_3D('',#198461,#120435,#120436);
#102146=AXIS2_PLACEMENT_3D('',#198462,#120437,#120438);
#102147=AXIS2_PLACEMENT_3D('',#198463,#120439,#120440);
#102148=AXIS2_PLACEMENT_3D('',#198464,#120441,#120442);
#102149=AXIS2_PLACEMENT_3D('',#198483,#120443,#120444);
#102150=AXIS2_PLACEMENT_3D('',#198484,#120445,#120446);
#102151=AXIS2_PLACEMENT_3D('',#198485,#120447,#120448);
#102152=AXIS2_PLACEMENT_3D('',#198486,#120449,#120450);
#102153=AXIS2_PLACEMENT_3D('',#198487,#120451,#120452);
#102154=AXIS2_PLACEMENT_3D('',#198500,#120453,#120454);
#102155=AXIS2_PLACEMENT_3D('',#198519,#120455,#120456);
#102156=AXIS2_PLACEMENT_3D('',#198520,#120457,#120458);
#102157=AXIS2_PLACEMENT_3D('',#198521,#120459,#120460);
#102158=AXIS2_PLACEMENT_3D('',#198522,#120461,#120462);
#102159=AXIS2_PLACEMENT_3D('',#198523,#120463,#120464);
#102160=AXIS2_PLACEMENT_3D('',#198542,#120465,#120466);
#102161=AXIS2_PLACEMENT_3D('',#198555,#120467,#120468);
#102162=AXIS2_PLACEMENT_3D('',#198556,#120469,#120470);
#102163=AXIS2_PLACEMENT_3D('',#198557,#120471,#120472);
#102164=AXIS2_PLACEMENT_3D('',#198558,#120473,#120474);
#102165=AXIS2_PLACEMENT_3D('',#198559,#120475,#120476);
#102166=AXIS2_PLACEMENT_3D('',#198578,#120477,#120478);
#102167=AXIS2_PLACEMENT_3D('',#198579,#120479,#120480);
#102168=AXIS2_PLACEMENT_3D('',#198580,#120481,#120482);
#102169=AXIS2_PLACEMENT_3D('',#198581,#120483,#120484);
#102170=AXIS2_PLACEMENT_3D('',#198582,#120485,#120486);
#102171=AXIS2_PLACEMENT_3D('',#198595,#120487,#120488);
#102172=AXIS2_PLACEMENT_3D('',#198608,#120489,#120490);
#102173=AXIS2_PLACEMENT_3D('',#198609,#120491,#120492);
#102174=AXIS2_PLACEMENT_3D('',#198610,#120493,#120494);
#102175=AXIS2_PLACEMENT_3D('',#198611,#120495,#120496);
#102176=AXIS2_PLACEMENT_3D('',#198612,#120497,#120498);
#102177=AXIS2_PLACEMENT_3D('',#198625,#120499,#120500);
#102178=AXIS2_PLACEMENT_3D('',#198626,#120501,#120502);
#102179=AXIS2_PLACEMENT_3D('',#198627,#120503,#120504);
#102180=AXIS2_PLACEMENT_3D('',#198628,#120505,#120506);
#102181=AXIS2_PLACEMENT_3D('',#198629,#120507,#120508);
#102182=AXIS2_PLACEMENT_3D('',#198642,#120509,#120510);
#102183=AXIS2_PLACEMENT_3D('',#198643,#120511,#120512);
#102184=AXIS2_PLACEMENT_3D('',#198644,#120513,#120514);
#102185=AXIS2_PLACEMENT_3D('',#198645,#120515,#120516);
#102186=AXIS2_PLACEMENT_3D('',#198646,#120517,#120518);
#102187=AXIS2_PLACEMENT_3D('',#198659,#120519,#120520);
#102188=AXIS2_PLACEMENT_3D('',#198672,#120521,#120522);
#102189=AXIS2_PLACEMENT_3D('',#198673,#120523,#120524);
#102190=AXIS2_PLACEMENT_3D('',#198674,#120525,#120526);
#102191=AXIS2_PLACEMENT_3D('',#198675,#120527,#120528);
#102192=AXIS2_PLACEMENT_3D('',#198676,#120529,#120530);
#102193=AXIS2_PLACEMENT_3D('',#198695,#120531,#120532);
#102194=AXIS2_PLACEMENT_3D('',#198696,#120533,#120534);
#102195=AXIS2_PLACEMENT_3D('',#198697,#120535,#120536);
#102196=AXIS2_PLACEMENT_3D('',#198698,#120537,#120538);
#102197=AXIS2_PLACEMENT_3D('',#198699,#120539,#120540);
#102198=AXIS2_PLACEMENT_3D('',#198712,#120541,#120542);
#102199=AXIS2_PLACEMENT_3D('',#198731,#120543,#120544);
#102200=AXIS2_PLACEMENT_3D('',#198732,#120545,#120546);
#102201=AXIS2_PLACEMENT_3D('',#198733,#120547,#120548);
#102202=AXIS2_PLACEMENT_3D('',#198734,#120549,#120550);
#102203=AXIS2_PLACEMENT_3D('',#198735,#120551,#120552);
#102204=AXIS2_PLACEMENT_3D('',#198754,#120553,#120554);
#102205=AXIS2_PLACEMENT_3D('',#198767,#120555,#120556);
#102206=AXIS2_PLACEMENT_3D('',#198768,#120557,#120558);
#102207=AXIS2_PLACEMENT_3D('',#198769,#120559,#120560);
#102208=AXIS2_PLACEMENT_3D('',#198770,#120561,#120562);
#102209=AXIS2_PLACEMENT_3D('',#198771,#120563,#120564);
#102210=AXIS2_PLACEMENT_3D('',#198790,#120565,#120566);
#102211=AXIS2_PLACEMENT_3D('',#198791,#120567,#120568);
#102212=AXIS2_PLACEMENT_3D('',#198792,#120569,#120570);
#102213=AXIS2_PLACEMENT_3D('',#198793,#120571,#120572);
#102214=AXIS2_PLACEMENT_3D('',#198794,#120573,#120574);
#102215=AXIS2_PLACEMENT_3D('',#198807,#120575,#120576);
#102216=AXIS2_PLACEMENT_3D('',#198820,#120577,#120578);
#102217=AXIS2_PLACEMENT_3D('',#198821,#120579,#120580);
#102218=AXIS2_PLACEMENT_3D('',#198822,#120581,#120582);
#102219=AXIS2_PLACEMENT_3D('',#198823,#120583,#120584);
#102220=AXIS2_PLACEMENT_3D('',#198824,#120585,#120586);
#102221=AXIS2_PLACEMENT_3D('',#198837,#120587,#120588);
#102222=AXIS2_PLACEMENT_3D('',#198838,#120589,#120590);
#102223=AXIS2_PLACEMENT_3D('',#198839,#120591,#120592);
#102224=AXIS2_PLACEMENT_3D('',#198840,#120593,#120594);
#102225=AXIS2_PLACEMENT_3D('',#198841,#120595,#120596);
#102226=AXIS2_PLACEMENT_3D('',#198854,#120597,#120598);
#102227=AXIS2_PLACEMENT_3D('',#198855,#120599,#120600);
#102228=AXIS2_PLACEMENT_3D('',#198856,#120601,#120602);
#102229=AXIS2_PLACEMENT_3D('',#198857,#120603,#120604);
#102230=AXIS2_PLACEMENT_3D('',#198858,#120605,#120606);
#102231=AXIS2_PLACEMENT_3D('',#198871,#120607,#120608);
#102232=AXIS2_PLACEMENT_3D('',#198884,#120609,#120610);
#102233=AXIS2_PLACEMENT_3D('',#198885,#120611,#120612);
#102234=AXIS2_PLACEMENT_3D('',#198886,#120613,#120614);
#102235=AXIS2_PLACEMENT_3D('',#198887,#120615,#120616);
#102236=AXIS2_PLACEMENT_3D('',#198888,#120617,#120618);
#102237=AXIS2_PLACEMENT_3D('',#198907,#120619,#120620);
#102238=AXIS2_PLACEMENT_3D('',#198908,#120621,#120622);
#102239=AXIS2_PLACEMENT_3D('',#198909,#120623,#120624);
#102240=AXIS2_PLACEMENT_3D('',#198910,#120625,#120626);
#102241=AXIS2_PLACEMENT_3D('',#198911,#120627,#120628);
#102242=AXIS2_PLACEMENT_3D('',#198924,#120629,#120630);
#102243=AXIS2_PLACEMENT_3D('',#198943,#120631,#120632);
#102244=AXIS2_PLACEMENT_3D('',#198944,#120633,#120634);
#102245=AXIS2_PLACEMENT_3D('',#198945,#120635,#120636);
#102246=AXIS2_PLACEMENT_3D('',#198946,#120637,#120638);
#102247=AXIS2_PLACEMENT_3D('',#198947,#120639,#120640);
#102248=AXIS2_PLACEMENT_3D('',#198966,#120641,#120642);
#102249=AXIS2_PLACEMENT_3D('',#198979,#120643,#120644);
#102250=AXIS2_PLACEMENT_3D('',#198980,#120645,#120646);
#102251=AXIS2_PLACEMENT_3D('',#198981,#120647,#120648);
#102252=AXIS2_PLACEMENT_3D('',#198982,#120649,#120650);
#102253=AXIS2_PLACEMENT_3D('',#198983,#120651,#120652);
#102254=AXIS2_PLACEMENT_3D('',#199002,#120653,#120654);
#102255=AXIS2_PLACEMENT_3D('',#199003,#120655,#120656);
#102256=AXIS2_PLACEMENT_3D('',#199004,#120657,#120658);
#102257=AXIS2_PLACEMENT_3D('',#199005,#120659,#120660);
#102258=AXIS2_PLACEMENT_3D('',#199006,#120661,#120662);
#102259=AXIS2_PLACEMENT_3D('',#199019,#120663,#120664);
#102260=AXIS2_PLACEMENT_3D('',#199032,#120665,#120666);
#102261=AXIS2_PLACEMENT_3D('',#199033,#120667,#120668);
#102262=AXIS2_PLACEMENT_3D('',#199034,#120669,#120670);
#102263=AXIS2_PLACEMENT_3D('',#199035,#120671,#120672);
#102264=AXIS2_PLACEMENT_3D('',#199036,#120673,#120674);
#102265=AXIS2_PLACEMENT_3D('',#199049,#120675,#120676);
#102266=AXIS2_PLACEMENT_3D('',#199050,#120677,#120678);
#102267=AXIS2_PLACEMENT_3D('',#199051,#120679,#120680);
#102268=AXIS2_PLACEMENT_3D('',#199052,#120681,#120682);
#102269=AXIS2_PLACEMENT_3D('',#199053,#120683,#120684);
#102270=AXIS2_PLACEMENT_3D('',#199066,#120685,#120686);
#102271=AXIS2_PLACEMENT_3D('',#199067,#120687,#120688);
#102272=AXIS2_PLACEMENT_3D('',#199068,#120689,#120690);
#102273=AXIS2_PLACEMENT_3D('',#199069,#120691,#120692);
#102274=AXIS2_PLACEMENT_3D('',#199070,#120693,#120694);
#102275=AXIS2_PLACEMENT_3D('',#199083,#120695,#120696);
#102276=AXIS2_PLACEMENT_3D('',#199096,#120697,#120698);
#102277=AXIS2_PLACEMENT_3D('',#199097,#120699,#120700);
#102278=AXIS2_PLACEMENT_3D('',#199098,#120701,#120702);
#102279=AXIS2_PLACEMENT_3D('',#199099,#120703,#120704);
#102280=AXIS2_PLACEMENT_3D('',#199100,#120705,#120706);
#102281=AXIS2_PLACEMENT_3D('',#199119,#120707,#120708);
#102282=AXIS2_PLACEMENT_3D('',#199120,#120709,#120710);
#102283=AXIS2_PLACEMENT_3D('',#199121,#120711,#120712);
#102284=AXIS2_PLACEMENT_3D('',#199122,#120713,#120714);
#102285=AXIS2_PLACEMENT_3D('',#199123,#120715,#120716);
#102286=AXIS2_PLACEMENT_3D('',#199136,#120717,#120718);
#102287=AXIS2_PLACEMENT_3D('',#199155,#120719,#120720);
#102288=AXIS2_PLACEMENT_3D('',#199156,#120721,#120722);
#102289=AXIS2_PLACEMENT_3D('',#199157,#120723,#120724);
#102290=AXIS2_PLACEMENT_3D('',#199158,#120725,#120726);
#102291=AXIS2_PLACEMENT_3D('',#199159,#120727,#120728);
#102292=AXIS2_PLACEMENT_3D('',#199178,#120729,#120730);
#102293=AXIS2_PLACEMENT_3D('',#199191,#120731,#120732);
#102294=AXIS2_PLACEMENT_3D('',#199192,#120733,#120734);
#102295=AXIS2_PLACEMENT_3D('',#199193,#120735,#120736);
#102296=AXIS2_PLACEMENT_3D('',#199194,#120737,#120738);
#102297=AXIS2_PLACEMENT_3D('',#199195,#120739,#120740);
#102298=AXIS2_PLACEMENT_3D('',#199214,#120741,#120742);
#102299=AXIS2_PLACEMENT_3D('',#199215,#120743,#120744);
#102300=AXIS2_PLACEMENT_3D('',#199216,#120745,#120746);
#102301=AXIS2_PLACEMENT_3D('',#199217,#120747,#120748);
#102302=AXIS2_PLACEMENT_3D('',#199218,#120749,#120750);
#102303=AXIS2_PLACEMENT_3D('',#199231,#120751,#120752);
#102304=AXIS2_PLACEMENT_3D('',#199244,#120753,#120754);
#102305=AXIS2_PLACEMENT_3D('',#199245,#120755,#120756);
#102306=AXIS2_PLACEMENT_3D('',#199246,#120757,#120758);
#102307=AXIS2_PLACEMENT_3D('',#199247,#120759,#120760);
#102308=AXIS2_PLACEMENT_3D('',#199248,#120761,#120762);
#102309=AXIS2_PLACEMENT_3D('',#199261,#120763,#120764);
#102310=AXIS2_PLACEMENT_3D('',#199262,#120765,#120766);
#102311=AXIS2_PLACEMENT_3D('',#199263,#120767,#120768);
#102312=AXIS2_PLACEMENT_3D('',#199264,#120769,#120770);
#102313=AXIS2_PLACEMENT_3D('',#199265,#120771,#120772);
#102314=AXIS2_PLACEMENT_3D('',#199278,#120773,#120774);
#102315=AXIS2_PLACEMENT_3D('',#199279,#120775,#120776);
#102316=AXIS2_PLACEMENT_3D('',#199280,#120777,#120778);
#102317=AXIS2_PLACEMENT_3D('',#199281,#120779,#120780);
#102318=AXIS2_PLACEMENT_3D('',#199282,#120781,#120782);
#102319=AXIS2_PLACEMENT_3D('',#199295,#120783,#120784);
#102320=AXIS2_PLACEMENT_3D('',#199308,#120785,#120786);
#102321=AXIS2_PLACEMENT_3D('',#199309,#120787,#120788);
#102322=AXIS2_PLACEMENT_3D('',#199310,#120789,#120790);
#102323=AXIS2_PLACEMENT_3D('',#199311,#120791,#120792);
#102324=AXIS2_PLACEMENT_3D('',#199312,#120793,#120794);
#102325=AXIS2_PLACEMENT_3D('',#199331,#120795,#120796);
#102326=AXIS2_PLACEMENT_3D('',#199332,#120797,#120798);
#102327=AXIS2_PLACEMENT_3D('',#199333,#120799,#120800);
#102328=AXIS2_PLACEMENT_3D('',#199334,#120801,#120802);
#102329=AXIS2_PLACEMENT_3D('',#199335,#120803,#120804);
#102330=AXIS2_PLACEMENT_3D('',#199348,#120805,#120806);
#102331=AXIS2_PLACEMENT_3D('',#199367,#120807,#120808);
#102332=AXIS2_PLACEMENT_3D('',#199368,#120809,#120810);
#102333=AXIS2_PLACEMENT_3D('',#199369,#120811,#120812);
#102334=AXIS2_PLACEMENT_3D('',#199370,#120813,#120814);
#102335=AXIS2_PLACEMENT_3D('',#199371,#120815,#120816);
#102336=AXIS2_PLACEMENT_3D('',#199390,#120817,#120818);
#102337=AXIS2_PLACEMENT_3D('',#199403,#120819,#120820);
#102338=AXIS2_PLACEMENT_3D('',#199404,#120821,#120822);
#102339=AXIS2_PLACEMENT_3D('',#199405,#120823,#120824);
#102340=AXIS2_PLACEMENT_3D('',#199406,#120825,#120826);
#102341=AXIS2_PLACEMENT_3D('',#199407,#120827,#120828);
#102342=AXIS2_PLACEMENT_3D('',#199426,#120829,#120830);
#102343=AXIS2_PLACEMENT_3D('',#199427,#120831,#120832);
#102344=AXIS2_PLACEMENT_3D('',#199428,#120833,#120834);
#102345=AXIS2_PLACEMENT_3D('',#199429,#120835,#120836);
#102346=AXIS2_PLACEMENT_3D('',#199430,#120837,#120838);
#102347=AXIS2_PLACEMENT_3D('',#199443,#120839,#120840);
#102348=AXIS2_PLACEMENT_3D('',#199456,#120841,#120842);
#102349=AXIS2_PLACEMENT_3D('',#199457,#120843,#120844);
#102350=AXIS2_PLACEMENT_3D('',#199458,#120845,#120846);
#102351=AXIS2_PLACEMENT_3D('',#199459,#120847,#120848);
#102352=AXIS2_PLACEMENT_3D('',#199460,#120849,#120850);
#102353=AXIS2_PLACEMENT_3D('',#199473,#120851,#120852);
#102354=AXIS2_PLACEMENT_3D('',#199474,#120853,#120854);
#102355=AXIS2_PLACEMENT_3D('',#199475,#120855,#120856);
#102356=AXIS2_PLACEMENT_3D('',#199476,#120857,#120858);
#102357=AXIS2_PLACEMENT_3D('',#199477,#120859,#120860);
#102358=AXIS2_PLACEMENT_3D('',#199490,#120861,#120862);
#102359=AXIS2_PLACEMENT_3D('',#199491,#120863,#120864);
#102360=AXIS2_PLACEMENT_3D('',#199492,#120865,#120866);
#102361=AXIS2_PLACEMENT_3D('',#199493,#120867,#120868);
#102362=AXIS2_PLACEMENT_3D('',#199494,#120869,#120870);
#102363=AXIS2_PLACEMENT_3D('',#199507,#120871,#120872);
#102364=AXIS2_PLACEMENT_3D('',#199520,#120873,#120874);
#102365=AXIS2_PLACEMENT_3D('',#199521,#120875,#120876);
#102366=AXIS2_PLACEMENT_3D('',#199522,#120877,#120878);
#102367=AXIS2_PLACEMENT_3D('',#199523,#120879,#120880);
#102368=AXIS2_PLACEMENT_3D('',#199524,#120881,#120882);
#102369=AXIS2_PLACEMENT_3D('',#199543,#120883,#120884);
#102370=AXIS2_PLACEMENT_3D('',#199544,#120885,#120886);
#102371=AXIS2_PLACEMENT_3D('',#199545,#120887,#120888);
#102372=AXIS2_PLACEMENT_3D('',#199546,#120889,#120890);
#102373=AXIS2_PLACEMENT_3D('',#199547,#120891,#120892);
#102374=AXIS2_PLACEMENT_3D('',#199560,#120893,#120894);
#102375=AXIS2_PLACEMENT_3D('',#199579,#120895,#120896);
#102376=AXIS2_PLACEMENT_3D('',#199580,#120897,#120898);
#102377=AXIS2_PLACEMENT_3D('',#199581,#120899,#120900);
#102378=AXIS2_PLACEMENT_3D('',#199582,#120901,#120902);
#102379=AXIS2_PLACEMENT_3D('',#199583,#120903,#120904);
#102380=AXIS2_PLACEMENT_3D('',#199602,#120905,#120906);
#102381=AXIS2_PLACEMENT_3D('',#199615,#120907,#120908);
#102382=AXIS2_PLACEMENT_3D('',#199616,#120909,#120910);
#102383=AXIS2_PLACEMENT_3D('',#199617,#120911,#120912);
#102384=AXIS2_PLACEMENT_3D('',#199618,#120913,#120914);
#102385=AXIS2_PLACEMENT_3D('',#199619,#120915,#120916);
#102386=AXIS2_PLACEMENT_3D('',#199638,#120917,#120918);
#102387=AXIS2_PLACEMENT_3D('',#199639,#120919,#120920);
#102388=AXIS2_PLACEMENT_3D('',#199640,#120921,#120922);
#102389=AXIS2_PLACEMENT_3D('',#199641,#120923,#120924);
#102390=AXIS2_PLACEMENT_3D('',#199642,#120925,#120926);
#102391=AXIS2_PLACEMENT_3D('',#199655,#120927,#120928);
#102392=AXIS2_PLACEMENT_3D('',#199668,#120929,#120930);
#102393=AXIS2_PLACEMENT_3D('',#199669,#120931,#120932);
#102394=AXIS2_PLACEMENT_3D('',#199670,#120933,#120934);
#102395=AXIS2_PLACEMENT_3D('',#199671,#120935,#120936);
#102396=AXIS2_PLACEMENT_3D('',#199672,#120937,#120938);
#102397=AXIS2_PLACEMENT_3D('',#199685,#120939,#120940);
#102398=AXIS2_PLACEMENT_3D('',#199686,#120941,#120942);
#102399=AXIS2_PLACEMENT_3D('',#199687,#120943,#120944);
#102400=AXIS2_PLACEMENT_3D('',#199688,#120945,#120946);
#102401=AXIS2_PLACEMENT_3D('',#199689,#120947,#120948);
#102402=AXIS2_PLACEMENT_3D('',#199702,#120949,#120950);
#102403=AXIS2_PLACEMENT_3D('',#199703,#120951,#120952);
#102404=AXIS2_PLACEMENT_3D('',#199704,#120953,#120954);
#102405=AXIS2_PLACEMENT_3D('',#199705,#120955,#120956);
#102406=AXIS2_PLACEMENT_3D('',#199706,#120957,#120958);
#102407=AXIS2_PLACEMENT_3D('',#199719,#120959,#120960);
#102408=AXIS2_PLACEMENT_3D('',#199732,#120961,#120962);
#102409=AXIS2_PLACEMENT_3D('',#199733,#120963,#120964);
#102410=AXIS2_PLACEMENT_3D('',#199734,#120965,#120966);
#102411=AXIS2_PLACEMENT_3D('',#199735,#120967,#120968);
#102412=AXIS2_PLACEMENT_3D('',#199736,#120969,#120970);
#102413=AXIS2_PLACEMENT_3D('',#199755,#120971,#120972);
#102414=AXIS2_PLACEMENT_3D('',#199756,#120973,#120974);
#102415=AXIS2_PLACEMENT_3D('',#199757,#120975,#120976);
#102416=AXIS2_PLACEMENT_3D('',#199758,#120977,#120978);
#102417=AXIS2_PLACEMENT_3D('',#199759,#120979,#120980);
#102418=AXIS2_PLACEMENT_3D('',#199772,#120981,#120982);
#102419=AXIS2_PLACEMENT_3D('',#199791,#120983,#120984);
#102420=AXIS2_PLACEMENT_3D('',#199792,#120985,#120986);
#102421=AXIS2_PLACEMENT_3D('',#199793,#120987,#120988);
#102422=AXIS2_PLACEMENT_3D('',#199794,#120989,#120990);
#102423=AXIS2_PLACEMENT_3D('',#199795,#120991,#120992);
#102424=AXIS2_PLACEMENT_3D('',#199814,#120993,#120994);
#102425=AXIS2_PLACEMENT_3D('',#199827,#120995,#120996);
#102426=AXIS2_PLACEMENT_3D('',#199828,#120997,#120998);
#102427=AXIS2_PLACEMENT_3D('',#199829,#120999,#121000);
#102428=AXIS2_PLACEMENT_3D('',#199830,#121001,#121002);
#102429=AXIS2_PLACEMENT_3D('',#199831,#121003,#121004);
#102430=AXIS2_PLACEMENT_3D('',#199850,#121005,#121006);
#102431=AXIS2_PLACEMENT_3D('',#199851,#121007,#121008);
#102432=AXIS2_PLACEMENT_3D('',#199852,#121009,#121010);
#102433=AXIS2_PLACEMENT_3D('',#199853,#121011,#121012);
#102434=AXIS2_PLACEMENT_3D('',#199854,#121013,#121014);
#102435=AXIS2_PLACEMENT_3D('',#199867,#121015,#121016);
#102436=AXIS2_PLACEMENT_3D('',#199880,#121017,#121018);
#102437=AXIS2_PLACEMENT_3D('',#199881,#121019,#121020);
#102438=AXIS2_PLACEMENT_3D('',#199882,#121021,#121022);
#102439=AXIS2_PLACEMENT_3D('',#199883,#121023,#121024);
#102440=AXIS2_PLACEMENT_3D('',#199884,#121025,#121026);
#102441=AXIS2_PLACEMENT_3D('',#199897,#121027,#121028);
#102442=AXIS2_PLACEMENT_3D('',#199898,#121029,#121030);
#102443=AXIS2_PLACEMENT_3D('',#199899,#121031,#121032);
#102444=AXIS2_PLACEMENT_3D('',#199900,#121033,#121034);
#102445=AXIS2_PLACEMENT_3D('',#199901,#121035,#121036);
#102446=AXIS2_PLACEMENT_3D('',#199914,#121037,#121038);
#102447=AXIS2_PLACEMENT_3D('',#199915,#121039,#121040);
#102448=AXIS2_PLACEMENT_3D('',#199916,#121041,#121042);
#102449=AXIS2_PLACEMENT_3D('',#199917,#121043,#121044);
#102450=AXIS2_PLACEMENT_3D('',#199918,#121045,#121046);
#102451=AXIS2_PLACEMENT_3D('',#199931,#121047,#121048);
#102452=AXIS2_PLACEMENT_3D('',#199944,#121049,#121050);
#102453=AXIS2_PLACEMENT_3D('',#199945,#121051,#121052);
#102454=AXIS2_PLACEMENT_3D('',#199946,#121053,#121054);
#102455=AXIS2_PLACEMENT_3D('',#199947,#121055,#121056);
#102456=AXIS2_PLACEMENT_3D('',#199948,#121057,#121058);
#102457=AXIS2_PLACEMENT_3D('',#199967,#121059,#121060);
#102458=AXIS2_PLACEMENT_3D('',#199968,#121061,#121062);
#102459=AXIS2_PLACEMENT_3D('',#199969,#121063,#121064);
#102460=AXIS2_PLACEMENT_3D('',#199970,#121065,#121066);
#102461=AXIS2_PLACEMENT_3D('',#199971,#121067,#121068);
#102462=AXIS2_PLACEMENT_3D('',#199984,#121069,#121070);
#102463=AXIS2_PLACEMENT_3D('',#200003,#121071,#121072);
#102464=AXIS2_PLACEMENT_3D('',#200004,#121073,#121074);
#102465=AXIS2_PLACEMENT_3D('',#200005,#121075,#121076);
#102466=AXIS2_PLACEMENT_3D('',#200006,#121077,#121078);
#102467=AXIS2_PLACEMENT_3D('',#200007,#121079,#121080);
#102468=AXIS2_PLACEMENT_3D('',#200026,#121081,#121082);
#102469=AXIS2_PLACEMENT_3D('',#200039,#121083,#121084);
#102470=AXIS2_PLACEMENT_3D('',#200040,#121085,#121086);
#102471=AXIS2_PLACEMENT_3D('',#200041,#121087,#121088);
#102472=AXIS2_PLACEMENT_3D('',#200042,#121089,#121090);
#102473=AXIS2_PLACEMENT_3D('',#200043,#121091,#121092);
#102474=AXIS2_PLACEMENT_3D('',#200062,#121093,#121094);
#102475=AXIS2_PLACEMENT_3D('',#200063,#121095,#121096);
#102476=AXIS2_PLACEMENT_3D('',#200064,#121097,#121098);
#102477=AXIS2_PLACEMENT_3D('',#200065,#121099,#121100);
#102478=AXIS2_PLACEMENT_3D('',#200066,#121101,#121102);
#102479=AXIS2_PLACEMENT_3D('',#200079,#121103,#121104);
#102480=AXIS2_PLACEMENT_3D('',#200092,#121105,#121106);
#102481=AXIS2_PLACEMENT_3D('',#200093,#121107,#121108);
#102482=AXIS2_PLACEMENT_3D('',#200094,#121109,#121110);
#102483=AXIS2_PLACEMENT_3D('',#200095,#121111,#121112);
#102484=AXIS2_PLACEMENT_3D('',#200096,#121113,#121114);
#102485=AXIS2_PLACEMENT_3D('',#200109,#121115,#121116);
#102486=AXIS2_PLACEMENT_3D('',#200110,#121117,#121118);
#102487=AXIS2_PLACEMENT_3D('',#200111,#121119,#121120);
#102488=AXIS2_PLACEMENT_3D('',#200112,#121121,#121122);
#102489=AXIS2_PLACEMENT_3D('',#200113,#121123,#121124);
#102490=AXIS2_PLACEMENT_3D('',#200126,#121125,#121126);
#102491=AXIS2_PLACEMENT_3D('',#200127,#121127,#121128);
#102492=AXIS2_PLACEMENT_3D('',#200128,#121129,#121130);
#102493=AXIS2_PLACEMENT_3D('',#200129,#121131,#121132);
#102494=AXIS2_PLACEMENT_3D('',#200130,#121133,#121134);
#102495=AXIS2_PLACEMENT_3D('',#200143,#121135,#121136);
#102496=AXIS2_PLACEMENT_3D('',#200156,#121137,#121138);
#102497=AXIS2_PLACEMENT_3D('',#200157,#121139,#121140);
#102498=AXIS2_PLACEMENT_3D('',#200158,#121141,#121142);
#102499=AXIS2_PLACEMENT_3D('',#200159,#121143,#121144);
#102500=AXIS2_PLACEMENT_3D('',#200160,#121145,#121146);
#102501=AXIS2_PLACEMENT_3D('',#200179,#121147,#121148);
#102502=AXIS2_PLACEMENT_3D('',#200180,#121149,#121150);
#102503=AXIS2_PLACEMENT_3D('',#200181,#121151,#121152);
#102504=AXIS2_PLACEMENT_3D('',#200182,#121153,#121154);
#102505=AXIS2_PLACEMENT_3D('',#200183,#121155,#121156);
#102506=AXIS2_PLACEMENT_3D('',#200196,#121157,#121158);
#102507=AXIS2_PLACEMENT_3D('',#200215,#121159,#121160);
#102508=AXIS2_PLACEMENT_3D('',#200216,#121161,#121162);
#102509=AXIS2_PLACEMENT_3D('',#200217,#121163,#121164);
#102510=AXIS2_PLACEMENT_3D('',#200218,#121165,#121166);
#102511=AXIS2_PLACEMENT_3D('',#200219,#121167,#121168);
#102512=AXIS2_PLACEMENT_3D('',#200238,#121169,#121170);
#102513=AXIS2_PLACEMENT_3D('',#200251,#121171,#121172);
#102514=AXIS2_PLACEMENT_3D('',#200252,#121173,#121174);
#102515=AXIS2_PLACEMENT_3D('',#200253,#121175,#121176);
#102516=AXIS2_PLACEMENT_3D('',#200254,#121177,#121178);
#102517=AXIS2_PLACEMENT_3D('',#200255,#121179,#121180);
#102518=AXIS2_PLACEMENT_3D('',#200274,#121181,#121182);
#102519=AXIS2_PLACEMENT_3D('',#200275,#121183,#121184);
#102520=AXIS2_PLACEMENT_3D('',#200276,#121185,#121186);
#102521=AXIS2_PLACEMENT_3D('',#200277,#121187,#121188);
#102522=AXIS2_PLACEMENT_3D('',#200278,#121189,#121190);
#102523=AXIS2_PLACEMENT_3D('',#200291,#121191,#121192);
#102524=AXIS2_PLACEMENT_3D('',#200304,#121193,#121194);
#102525=AXIS2_PLACEMENT_3D('',#200305,#121195,#121196);
#102526=AXIS2_PLACEMENT_3D('',#200306,#121197,#121198);
#102527=AXIS2_PLACEMENT_3D('',#200307,#121199,#121200);
#102528=AXIS2_PLACEMENT_3D('',#200308,#121201,#121202);
#102529=AXIS2_PLACEMENT_3D('',#200321,#121203,#121204);
#102530=AXIS2_PLACEMENT_3D('',#200322,#121205,#121206);
#102531=AXIS2_PLACEMENT_3D('',#200323,#121207,#121208);
#102532=AXIS2_PLACEMENT_3D('',#200324,#121209,#121210);
#102533=AXIS2_PLACEMENT_3D('',#200325,#121211,#121212);
#102534=AXIS2_PLACEMENT_3D('',#200338,#121213,#121214);
#102535=AXIS2_PLACEMENT_3D('',#200339,#121215,#121216);
#102536=AXIS2_PLACEMENT_3D('',#200340,#121217,#121218);
#102537=AXIS2_PLACEMENT_3D('',#200341,#121219,#121220);
#102538=AXIS2_PLACEMENT_3D('',#200342,#121221,#121222);
#102539=AXIS2_PLACEMENT_3D('',#200355,#121223,#121224);
#102540=AXIS2_PLACEMENT_3D('',#200368,#121225,#121226);
#102541=AXIS2_PLACEMENT_3D('',#200369,#121227,#121228);
#102542=AXIS2_PLACEMENT_3D('',#200370,#121229,#121230);
#102543=AXIS2_PLACEMENT_3D('',#200371,#121231,#121232);
#102544=AXIS2_PLACEMENT_3D('',#200372,#121233,#121234);
#102545=AXIS2_PLACEMENT_3D('',#200391,#121235,#121236);
#102546=AXIS2_PLACEMENT_3D('',#200392,#121237,#121238);
#102547=AXIS2_PLACEMENT_3D('',#200393,#121239,#121240);
#102548=AXIS2_PLACEMENT_3D('',#200394,#121241,#121242);
#102549=AXIS2_PLACEMENT_3D('',#200395,#121243,#121244);
#102550=AXIS2_PLACEMENT_3D('',#200408,#121245,#121246);
#102551=AXIS2_PLACEMENT_3D('',#200427,#121247,#121248);
#102552=AXIS2_PLACEMENT_3D('',#200428,#121249,#121250);
#102553=AXIS2_PLACEMENT_3D('',#200429,#121251,#121252);
#102554=AXIS2_PLACEMENT_3D('',#200430,#121253,#121254);
#102555=AXIS2_PLACEMENT_3D('',#200431,#121255,#121256);
#102556=AXIS2_PLACEMENT_3D('',#200450,#121257,#121258);
#102557=AXIS2_PLACEMENT_3D('',#200463,#121259,#121260);
#102558=AXIS2_PLACEMENT_3D('',#200464,#121261,#121262);
#102559=AXIS2_PLACEMENT_3D('',#200465,#121263,#121264);
#102560=AXIS2_PLACEMENT_3D('',#200466,#121265,#121266);
#102561=AXIS2_PLACEMENT_3D('',#200467,#121267,#121268);
#102562=AXIS2_PLACEMENT_3D('',#200486,#121269,#121270);
#102563=AXIS2_PLACEMENT_3D('',#200487,#121271,#121272);
#102564=AXIS2_PLACEMENT_3D('',#200488,#121273,#121274);
#102565=AXIS2_PLACEMENT_3D('',#200489,#121275,#121276);
#102566=AXIS2_PLACEMENT_3D('',#200490,#121277,#121278);
#102567=AXIS2_PLACEMENT_3D('',#200503,#121279,#121280);
#102568=AXIS2_PLACEMENT_3D('',#200516,#121281,#121282);
#102569=AXIS2_PLACEMENT_3D('',#200517,#121283,#121284);
#102570=AXIS2_PLACEMENT_3D('',#200518,#121285,#121286);
#102571=AXIS2_PLACEMENT_3D('',#200519,#121287,#121288);
#102572=AXIS2_PLACEMENT_3D('',#200520,#121289,#121290);
#102573=AXIS2_PLACEMENT_3D('',#200533,#121291,#121292);
#102574=AXIS2_PLACEMENT_3D('',#200534,#121293,#121294);
#102575=AXIS2_PLACEMENT_3D('',#200535,#121295,#121296);
#102576=AXIS2_PLACEMENT_3D('',#200536,#121297,#121298);
#102577=AXIS2_PLACEMENT_3D('',#200537,#121299,#121300);
#102578=AXIS2_PLACEMENT_3D('',#200550,#121301,#121302);
#102579=AXIS2_PLACEMENT_3D('',#200551,#121303,#121304);
#102580=AXIS2_PLACEMENT_3D('',#200552,#121305,#121306);
#102581=AXIS2_PLACEMENT_3D('',#200553,#121307,#121308);
#102582=AXIS2_PLACEMENT_3D('',#200554,#121309,#121310);
#102583=AXIS2_PLACEMENT_3D('',#200567,#121311,#121312);
#102584=AXIS2_PLACEMENT_3D('',#200580,#121313,#121314);
#102585=AXIS2_PLACEMENT_3D('',#200581,#121315,#121316);
#102586=AXIS2_PLACEMENT_3D('',#200582,#121317,#121318);
#102587=AXIS2_PLACEMENT_3D('',#200583,#121319,#121320);
#102588=AXIS2_PLACEMENT_3D('',#200584,#121321,#121322);
#102589=AXIS2_PLACEMENT_3D('',#200603,#121323,#121324);
#102590=AXIS2_PLACEMENT_3D('',#200604,#121325,#121326);
#102591=AXIS2_PLACEMENT_3D('',#200605,#121327,#121328);
#102592=AXIS2_PLACEMENT_3D('',#200606,#121329,#121330);
#102593=AXIS2_PLACEMENT_3D('',#200607,#121331,#121332);
#102594=AXIS2_PLACEMENT_3D('',#200620,#121333,#121334);
#102595=AXIS2_PLACEMENT_3D('',#200639,#121335,#121336);
#102596=AXIS2_PLACEMENT_3D('',#200640,#121337,#121338);
#102597=AXIS2_PLACEMENT_3D('',#200641,#121339,#121340);
#102598=AXIS2_PLACEMENT_3D('',#200642,#121341,#121342);
#102599=AXIS2_PLACEMENT_3D('',#200643,#121343,#121344);
#102600=AXIS2_PLACEMENT_3D('',#200662,#121345,#121346);
#102601=AXIS2_PLACEMENT_3D('',#200675,#121347,#121348);
#102602=AXIS2_PLACEMENT_3D('',#200676,#121349,#121350);
#102603=AXIS2_PLACEMENT_3D('',#200677,#121351,#121352);
#102604=AXIS2_PLACEMENT_3D('',#200678,#121353,#121354);
#102605=AXIS2_PLACEMENT_3D('',#200679,#121355,#121356);
#102606=AXIS2_PLACEMENT_3D('',#200698,#121357,#121358);
#102607=AXIS2_PLACEMENT_3D('',#200699,#121359,#121360);
#102608=AXIS2_PLACEMENT_3D('',#200700,#121361,#121362);
#102609=AXIS2_PLACEMENT_3D('',#200701,#121363,#121364);
#102610=AXIS2_PLACEMENT_3D('',#200702,#121365,#121366);
#102611=AXIS2_PLACEMENT_3D('',#200715,#121367,#121368);
#102612=AXIS2_PLACEMENT_3D('',#200728,#121369,#121370);
#102613=AXIS2_PLACEMENT_3D('',#200729,#121371,#121372);
#102614=AXIS2_PLACEMENT_3D('',#200730,#121373,#121374);
#102615=AXIS2_PLACEMENT_3D('',#200731,#121375,#121376);
#102616=AXIS2_PLACEMENT_3D('',#200732,#121377,#121378);
#102617=AXIS2_PLACEMENT_3D('',#200745,#121379,#121380);
#102618=AXIS2_PLACEMENT_3D('',#200746,#121381,#121382);
#102619=AXIS2_PLACEMENT_3D('',#200747,#121383,#121384);
#102620=AXIS2_PLACEMENT_3D('',#200748,#121385,#121386);
#102621=AXIS2_PLACEMENT_3D('',#200749,#121387,#121388);
#102622=AXIS2_PLACEMENT_3D('',#200762,#121389,#121390);
#102623=AXIS2_PLACEMENT_3D('',#200763,#121391,#121392);
#102624=AXIS2_PLACEMENT_3D('',#200764,#121393,#121394);
#102625=AXIS2_PLACEMENT_3D('',#200765,#121395,#121396);
#102626=AXIS2_PLACEMENT_3D('',#200766,#121397,#121398);
#102627=AXIS2_PLACEMENT_3D('',#200779,#121399,#121400);
#102628=AXIS2_PLACEMENT_3D('',#200792,#121401,#121402);
#102629=AXIS2_PLACEMENT_3D('',#200793,#121403,#121404);
#102630=AXIS2_PLACEMENT_3D('',#200794,#121405,#121406);
#102631=AXIS2_PLACEMENT_3D('',#200795,#121407,#121408);
#102632=AXIS2_PLACEMENT_3D('',#200796,#121409,#121410);
#102633=AXIS2_PLACEMENT_3D('',#200815,#121411,#121412);
#102634=AXIS2_PLACEMENT_3D('',#200816,#121413,#121414);
#102635=AXIS2_PLACEMENT_3D('',#200817,#121415,#121416);
#102636=AXIS2_PLACEMENT_3D('',#200818,#121417,#121418);
#102637=AXIS2_PLACEMENT_3D('',#200819,#121419,#121420);
#102638=AXIS2_PLACEMENT_3D('',#200832,#121421,#121422);
#102639=AXIS2_PLACEMENT_3D('',#200851,#121423,#121424);
#102640=AXIS2_PLACEMENT_3D('',#200852,#121425,#121426);
#102641=AXIS2_PLACEMENT_3D('',#200853,#121427,#121428);
#102642=AXIS2_PLACEMENT_3D('',#200854,#121429,#121430);
#102643=AXIS2_PLACEMENT_3D('',#200855,#121431,#121432);
#102644=AXIS2_PLACEMENT_3D('',#200874,#121433,#121434);
#102645=AXIS2_PLACEMENT_3D('',#200887,#121435,#121436);
#102646=AXIS2_PLACEMENT_3D('',#200888,#121437,#121438);
#102647=AXIS2_PLACEMENT_3D('',#200889,#121439,#121440);
#102648=AXIS2_PLACEMENT_3D('',#200890,#121441,#121442);
#102649=AXIS2_PLACEMENT_3D('',#200891,#121443,#121444);
#102650=AXIS2_PLACEMENT_3D('',#200910,#121445,#121446);
#102651=AXIS2_PLACEMENT_3D('',#200911,#121447,#121448);
#102652=AXIS2_PLACEMENT_3D('',#200912,#121449,#121450);
#102653=AXIS2_PLACEMENT_3D('',#200913,#121451,#121452);
#102654=AXIS2_PLACEMENT_3D('',#200914,#121453,#121454);
#102655=AXIS2_PLACEMENT_3D('',#200927,#121455,#121456);
#102656=AXIS2_PLACEMENT_3D('',#200940,#121457,#121458);
#102657=AXIS2_PLACEMENT_3D('',#200941,#121459,#121460);
#102658=AXIS2_PLACEMENT_3D('',#200942,#121461,#121462);
#102659=AXIS2_PLACEMENT_3D('',#200943,#121463,#121464);
#102660=AXIS2_PLACEMENT_3D('',#200944,#121465,#121466);
#102661=AXIS2_PLACEMENT_3D('',#200957,#121467,#121468);
#102662=AXIS2_PLACEMENT_3D('',#200958,#121469,#121470);
#102663=AXIS2_PLACEMENT_3D('',#200959,#121471,#121472);
#102664=AXIS2_PLACEMENT_3D('',#200960,#121473,#121474);
#102665=AXIS2_PLACEMENT_3D('',#200961,#121475,#121476);
#102666=AXIS2_PLACEMENT_3D('',#200974,#121477,#121478);
#102667=AXIS2_PLACEMENT_3D('',#200975,#121479,#121480);
#102668=AXIS2_PLACEMENT_3D('',#200976,#121481,#121482);
#102669=AXIS2_PLACEMENT_3D('',#200977,#121483,#121484);
#102670=AXIS2_PLACEMENT_3D('',#200978,#121485,#121486);
#102671=AXIS2_PLACEMENT_3D('',#200991,#121487,#121488);
#102672=AXIS2_PLACEMENT_3D('',#201004,#121489,#121490);
#102673=AXIS2_PLACEMENT_3D('',#201005,#121491,#121492);
#102674=AXIS2_PLACEMENT_3D('',#201006,#121493,#121494);
#102675=AXIS2_PLACEMENT_3D('',#201007,#121495,#121496);
#102676=AXIS2_PLACEMENT_3D('',#201008,#121497,#121498);
#102677=AXIS2_PLACEMENT_3D('',#201027,#121499,#121500);
#102678=AXIS2_PLACEMENT_3D('',#201028,#121501,#121502);
#102679=AXIS2_PLACEMENT_3D('',#201029,#121503,#121504);
#102680=AXIS2_PLACEMENT_3D('',#201030,#121505,#121506);
#102681=AXIS2_PLACEMENT_3D('',#201031,#121507,#121508);
#102682=AXIS2_PLACEMENT_3D('',#201044,#121509,#121510);
#102683=AXIS2_PLACEMENT_3D('',#201063,#121511,#121512);
#102684=AXIS2_PLACEMENT_3D('',#201064,#121513,#121514);
#102685=AXIS2_PLACEMENT_3D('',#201065,#121515,#121516);
#102686=AXIS2_PLACEMENT_3D('',#201066,#121517,#121518);
#102687=AXIS2_PLACEMENT_3D('',#201067,#121519,#121520);
#102688=AXIS2_PLACEMENT_3D('',#201086,#121521,#121522);
#102689=AXIS2_PLACEMENT_3D('',#201099,#121523,#121524);
#102690=AXIS2_PLACEMENT_3D('',#201100,#121525,#121526);
#102691=AXIS2_PLACEMENT_3D('',#201101,#121527,#121528);
#102692=AXIS2_PLACEMENT_3D('',#201102,#121529,#121530);
#102693=AXIS2_PLACEMENT_3D('',#201103,#121531,#121532);
#102694=AXIS2_PLACEMENT_3D('',#201122,#121533,#121534);
#102695=AXIS2_PLACEMENT_3D('',#201123,#121535,#121536);
#102696=AXIS2_PLACEMENT_3D('',#201124,#121537,#121538);
#102697=AXIS2_PLACEMENT_3D('',#201125,#121539,#121540);
#102698=AXIS2_PLACEMENT_3D('',#201126,#121541,#121542);
#102699=AXIS2_PLACEMENT_3D('',#201139,#121543,#121544);
#102700=AXIS2_PLACEMENT_3D('',#201152,#121545,#121546);
#102701=AXIS2_PLACEMENT_3D('',#201153,#121547,#121548);
#102702=AXIS2_PLACEMENT_3D('',#201154,#121549,#121550);
#102703=AXIS2_PLACEMENT_3D('',#201155,#121551,#121552);
#102704=AXIS2_PLACEMENT_3D('',#201156,#121553,#121554);
#102705=AXIS2_PLACEMENT_3D('',#201169,#121555,#121556);
#102706=AXIS2_PLACEMENT_3D('',#201170,#121557,#121558);
#102707=AXIS2_PLACEMENT_3D('',#201171,#121559,#121560);
#102708=AXIS2_PLACEMENT_3D('',#201172,#121561,#121562);
#102709=AXIS2_PLACEMENT_3D('',#201173,#121563,#121564);
#102710=AXIS2_PLACEMENT_3D('',#201186,#121565,#121566);
#102711=AXIS2_PLACEMENT_3D('',#201187,#121567,#121568);
#102712=AXIS2_PLACEMENT_3D('',#201188,#121569,#121570);
#102713=AXIS2_PLACEMENT_3D('',#201189,#121571,#121572);
#102714=AXIS2_PLACEMENT_3D('',#201190,#121573,#121574);
#102715=AXIS2_PLACEMENT_3D('',#201203,#121575,#121576);
#102716=AXIS2_PLACEMENT_3D('',#201216,#121577,#121578);
#102717=AXIS2_PLACEMENT_3D('',#201217,#121579,#121580);
#102718=AXIS2_PLACEMENT_3D('',#201218,#121581,#121582);
#102719=AXIS2_PLACEMENT_3D('',#201219,#121583,#121584);
#102720=AXIS2_PLACEMENT_3D('',#201220,#121585,#121586);
#102721=AXIS2_PLACEMENT_3D('',#201239,#121587,#121588);
#102722=AXIS2_PLACEMENT_3D('',#201240,#121589,#121590);
#102723=AXIS2_PLACEMENT_3D('',#201241,#121591,#121592);
#102724=AXIS2_PLACEMENT_3D('',#201242,#121593,#121594);
#102725=AXIS2_PLACEMENT_3D('',#201243,#121595,#121596);
#102726=AXIS2_PLACEMENT_3D('',#201256,#121597,#121598);
#102727=AXIS2_PLACEMENT_3D('',#201275,#121599,#121600);
#102728=AXIS2_PLACEMENT_3D('',#201276,#121601,#121602);
#102729=AXIS2_PLACEMENT_3D('',#201277,#121603,#121604);
#102730=AXIS2_PLACEMENT_3D('',#201278,#121605,#121606);
#102731=AXIS2_PLACEMENT_3D('',#201279,#121607,#121608);
#102732=AXIS2_PLACEMENT_3D('',#201298,#121609,#121610);
#102733=AXIS2_PLACEMENT_3D('',#201311,#121611,#121612);
#102734=AXIS2_PLACEMENT_3D('',#201312,#121613,#121614);
#102735=AXIS2_PLACEMENT_3D('',#201313,#121615,#121616);
#102736=AXIS2_PLACEMENT_3D('',#201314,#121617,#121618);
#102737=AXIS2_PLACEMENT_3D('',#201315,#121619,#121620);
#102738=AXIS2_PLACEMENT_3D('',#201334,#121621,#121622);
#102739=AXIS2_PLACEMENT_3D('',#201335,#121623,#121624);
#102740=AXIS2_PLACEMENT_3D('',#201336,#121625,#121626);
#102741=AXIS2_PLACEMENT_3D('',#201337,#121627,#121628);
#102742=AXIS2_PLACEMENT_3D('',#201338,#121629,#121630);
#102743=AXIS2_PLACEMENT_3D('',#201351,#121631,#121632);
#102744=AXIS2_PLACEMENT_3D('',#201364,#121633,#121634);
#102745=AXIS2_PLACEMENT_3D('',#201365,#121635,#121636);
#102746=AXIS2_PLACEMENT_3D('',#201366,#121637,#121638);
#102747=AXIS2_PLACEMENT_3D('',#201367,#121639,#121640);
#102748=AXIS2_PLACEMENT_3D('',#201368,#121641,#121642);
#102749=AXIS2_PLACEMENT_3D('',#201381,#121643,#121644);
#102750=AXIS2_PLACEMENT_3D('',#201382,#121645,#121646);
#102751=AXIS2_PLACEMENT_3D('',#201383,#121647,#121648);
#102752=AXIS2_PLACEMENT_3D('',#201384,#121649,#121650);
#102753=AXIS2_PLACEMENT_3D('',#201385,#121651,#121652);
#102754=AXIS2_PLACEMENT_3D('',#201398,#121653,#121654);
#102755=AXIS2_PLACEMENT_3D('',#201399,#121655,#121656);
#102756=AXIS2_PLACEMENT_3D('',#201400,#121657,#121658);
#102757=AXIS2_PLACEMENT_3D('',#201401,#121659,#121660);
#102758=AXIS2_PLACEMENT_3D('',#201402,#121661,#121662);
#102759=AXIS2_PLACEMENT_3D('',#201415,#121663,#121664);
#102760=AXIS2_PLACEMENT_3D('',#201428,#121665,#121666);
#102761=AXIS2_PLACEMENT_3D('',#201429,#121667,#121668);
#102762=AXIS2_PLACEMENT_3D('',#201430,#121669,#121670);
#102763=AXIS2_PLACEMENT_3D('',#201431,#121671,#121672);
#102764=AXIS2_PLACEMENT_3D('',#201432,#121673,#121674);
#102765=AXIS2_PLACEMENT_3D('',#201451,#121675,#121676);
#102766=AXIS2_PLACEMENT_3D('',#201452,#121677,#121678);
#102767=AXIS2_PLACEMENT_3D('',#201453,#121679,#121680);
#102768=AXIS2_PLACEMENT_3D('',#201454,#121681,#121682);
#102769=AXIS2_PLACEMENT_3D('',#201455,#121683,#121684);
#102770=AXIS2_PLACEMENT_3D('',#201468,#121685,#121686);
#102771=AXIS2_PLACEMENT_3D('',#201487,#121687,#121688);
#102772=AXIS2_PLACEMENT_3D('',#201488,#121689,#121690);
#102773=AXIS2_PLACEMENT_3D('',#201489,#121691,#121692);
#102774=AXIS2_PLACEMENT_3D('',#201490,#121693,#121694);
#102775=AXIS2_PLACEMENT_3D('',#201491,#121695,#121696);
#102776=AXIS2_PLACEMENT_3D('',#201510,#121697,#121698);
#102777=AXIS2_PLACEMENT_3D('',#201523,#121699,#121700);
#102778=AXIS2_PLACEMENT_3D('',#201524,#121701,#121702);
#102779=AXIS2_PLACEMENT_3D('',#201525,#121703,#121704);
#102780=AXIS2_PLACEMENT_3D('',#201526,#121705,#121706);
#102781=AXIS2_PLACEMENT_3D('',#201527,#121707,#121708);
#102782=AXIS2_PLACEMENT_3D('',#201546,#121709,#121710);
#102783=AXIS2_PLACEMENT_3D('',#201547,#121711,#121712);
#102784=AXIS2_PLACEMENT_3D('',#201548,#121713,#121714);
#102785=AXIS2_PLACEMENT_3D('',#201549,#121715,#121716);
#102786=AXIS2_PLACEMENT_3D('',#201550,#121717,#121718);
#102787=AXIS2_PLACEMENT_3D('',#201563,#121719,#121720);
#102788=AXIS2_PLACEMENT_3D('',#201576,#121721,#121722);
#102789=AXIS2_PLACEMENT_3D('',#201577,#121723,#121724);
#102790=AXIS2_PLACEMENT_3D('',#201578,#121725,#121726);
#102791=AXIS2_PLACEMENT_3D('',#201579,#121727,#121728);
#102792=AXIS2_PLACEMENT_3D('',#201580,#121729,#121730);
#102793=AXIS2_PLACEMENT_3D('',#201593,#121731,#121732);
#102794=AXIS2_PLACEMENT_3D('',#201594,#121733,#121734);
#102795=AXIS2_PLACEMENT_3D('',#201595,#121735,#121736);
#102796=AXIS2_PLACEMENT_3D('',#201596,#121737,#121738);
#102797=AXIS2_PLACEMENT_3D('',#201597,#121739,#121740);
#102798=AXIS2_PLACEMENT_3D('',#201610,#121741,#121742);
#102799=AXIS2_PLACEMENT_3D('',#201611,#121743,#121744);
#102800=AXIS2_PLACEMENT_3D('',#201612,#121745,#121746);
#102801=AXIS2_PLACEMENT_3D('',#201613,#121747,#121748);
#102802=AXIS2_PLACEMENT_3D('',#201614,#121749,#121750);
#102803=AXIS2_PLACEMENT_3D('',#201627,#121751,#121752);
#102804=AXIS2_PLACEMENT_3D('',#201640,#121753,#121754);
#102805=AXIS2_PLACEMENT_3D('',#201641,#121755,#121756);
#102806=AXIS2_PLACEMENT_3D('',#201642,#121757,#121758);
#102807=AXIS2_PLACEMENT_3D('',#201643,#121759,#121760);
#102808=AXIS2_PLACEMENT_3D('',#201644,#121761,#121762);
#102809=AXIS2_PLACEMENT_3D('',#201663,#121763,#121764);
#102810=AXIS2_PLACEMENT_3D('',#201664,#121765,#121766);
#102811=AXIS2_PLACEMENT_3D('',#201665,#121767,#121768);
#102812=AXIS2_PLACEMENT_3D('',#201666,#121769,#121770);
#102813=AXIS2_PLACEMENT_3D('',#201667,#121771,#121772);
#102814=AXIS2_PLACEMENT_3D('',#201680,#121773,#121774);
#102815=AXIS2_PLACEMENT_3D('',#201699,#121775,#121776);
#102816=AXIS2_PLACEMENT_3D('',#201700,#121777,#121778);
#102817=AXIS2_PLACEMENT_3D('',#201701,#121779,#121780);
#102818=AXIS2_PLACEMENT_3D('',#201702,#121781,#121782);
#102819=AXIS2_PLACEMENT_3D('',#201703,#121783,#121784);
#102820=AXIS2_PLACEMENT_3D('',#201722,#121785,#121786);
#102821=AXIS2_PLACEMENT_3D('',#201735,#121787,#121788);
#102822=AXIS2_PLACEMENT_3D('',#201736,#121789,#121790);
#102823=AXIS2_PLACEMENT_3D('',#201737,#121791,#121792);
#102824=AXIS2_PLACEMENT_3D('',#201738,#121793,#121794);
#102825=AXIS2_PLACEMENT_3D('',#201739,#121795,#121796);
#102826=AXIS2_PLACEMENT_3D('',#201758,#121797,#121798);
#102827=AXIS2_PLACEMENT_3D('',#201759,#121799,#121800);
#102828=AXIS2_PLACEMENT_3D('',#201760,#121801,#121802);
#102829=AXIS2_PLACEMENT_3D('',#201761,#121803,#121804);
#102830=AXIS2_PLACEMENT_3D('',#201762,#121805,#121806);
#102831=AXIS2_PLACEMENT_3D('',#201775,#121807,#121808);
#102832=AXIS2_PLACEMENT_3D('',#201788,#121809,#121810);
#102833=AXIS2_PLACEMENT_3D('',#201789,#121811,#121812);
#102834=AXIS2_PLACEMENT_3D('',#201790,#121813,#121814);
#102835=AXIS2_PLACEMENT_3D('',#201791,#121815,#121816);
#102836=AXIS2_PLACEMENT_3D('',#201792,#121817,#121818);
#102837=AXIS2_PLACEMENT_3D('',#201805,#121819,#121820);
#102838=AXIS2_PLACEMENT_3D('',#201806,#121821,#121822);
#102839=AXIS2_PLACEMENT_3D('',#201807,#121823,#121824);
#102840=AXIS2_PLACEMENT_3D('',#201808,#121825,#121826);
#102841=AXIS2_PLACEMENT_3D('',#201809,#121827,#121828);
#102842=AXIS2_PLACEMENT_3D('',#201822,#121829,#121830);
#102843=AXIS2_PLACEMENT_3D('',#201823,#121831,#121832);
#102844=AXIS2_PLACEMENT_3D('',#201824,#121833,#121834);
#102845=AXIS2_PLACEMENT_3D('',#201825,#121835,#121836);
#102846=AXIS2_PLACEMENT_3D('',#201826,#121837,#121838);
#102847=AXIS2_PLACEMENT_3D('',#201839,#121839,#121840);
#102848=AXIS2_PLACEMENT_3D('',#201852,#121841,#121842);
#102849=AXIS2_PLACEMENT_3D('',#201853,#121843,#121844);
#102850=AXIS2_PLACEMENT_3D('',#201854,#121845,#121846);
#102851=AXIS2_PLACEMENT_3D('',#201855,#121847,#121848);
#102852=AXIS2_PLACEMENT_3D('',#201856,#121849,#121850);
#102853=AXIS2_PLACEMENT_3D('',#201875,#121851,#121852);
#102854=AXIS2_PLACEMENT_3D('',#201876,#121853,#121854);
#102855=AXIS2_PLACEMENT_3D('',#201877,#121855,#121856);
#102856=AXIS2_PLACEMENT_3D('',#201878,#121857,#121858);
#102857=AXIS2_PLACEMENT_3D('',#201879,#121859,#121860);
#102858=AXIS2_PLACEMENT_3D('',#201892,#121861,#121862);
#102859=AXIS2_PLACEMENT_3D('',#201911,#121863,#121864);
#102860=AXIS2_PLACEMENT_3D('',#201912,#121865,#121866);
#102861=AXIS2_PLACEMENT_3D('',#201913,#121867,#121868);
#102862=AXIS2_PLACEMENT_3D('',#201914,#121869,#121870);
#102863=AXIS2_PLACEMENT_3D('',#201915,#121871,#121872);
#102864=AXIS2_PLACEMENT_3D('',#201934,#121873,#121874);
#102865=AXIS2_PLACEMENT_3D('',#201947,#121875,#121876);
#102866=AXIS2_PLACEMENT_3D('',#201948,#121877,#121878);
#102867=AXIS2_PLACEMENT_3D('',#201949,#121879,#121880);
#102868=AXIS2_PLACEMENT_3D('',#201950,#121881,#121882);
#102869=AXIS2_PLACEMENT_3D('',#201951,#121883,#121884);
#102870=AXIS2_PLACEMENT_3D('',#201970,#121885,#121886);
#102871=AXIS2_PLACEMENT_3D('',#201971,#121887,#121888);
#102872=AXIS2_PLACEMENT_3D('',#201972,#121889,#121890);
#102873=AXIS2_PLACEMENT_3D('',#201973,#121891,#121892);
#102874=AXIS2_PLACEMENT_3D('',#201974,#121893,#121894);
#102875=AXIS2_PLACEMENT_3D('',#201987,#121895,#121896);
#102876=AXIS2_PLACEMENT_3D('',#202000,#121897,#121898);
#102877=AXIS2_PLACEMENT_3D('',#202001,#121899,#121900);
#102878=AXIS2_PLACEMENT_3D('',#202002,#121901,#121902);
#102879=AXIS2_PLACEMENT_3D('',#202003,#121903,#121904);
#102880=AXIS2_PLACEMENT_3D('',#202004,#121905,#121906);
#102881=AXIS2_PLACEMENT_3D('',#202017,#121907,#121908);
#102882=AXIS2_PLACEMENT_3D('',#202018,#121909,#121910);
#102883=AXIS2_PLACEMENT_3D('',#202019,#121911,#121912);
#102884=AXIS2_PLACEMENT_3D('',#202020,#121913,#121914);
#102885=AXIS2_PLACEMENT_3D('',#202021,#121915,#121916);
#102886=AXIS2_PLACEMENT_3D('',#202034,#121917,#121918);
#102887=AXIS2_PLACEMENT_3D('',#202035,#121919,#121920);
#102888=AXIS2_PLACEMENT_3D('',#202036,#121921,#121922);
#102889=AXIS2_PLACEMENT_3D('',#202037,#121923,#121924);
#102890=AXIS2_PLACEMENT_3D('',#202038,#121925,#121926);
#102891=AXIS2_PLACEMENT_3D('',#202051,#121927,#121928);
#102892=AXIS2_PLACEMENT_3D('',#202064,#121929,#121930);
#102893=AXIS2_PLACEMENT_3D('',#202065,#121931,#121932);
#102894=AXIS2_PLACEMENT_3D('',#202066,#121933,#121934);
#102895=AXIS2_PLACEMENT_3D('',#202067,#121935,#121936);
#102896=AXIS2_PLACEMENT_3D('',#202068,#121937,#121938);
#102897=AXIS2_PLACEMENT_3D('',#202087,#121939,#121940);
#102898=AXIS2_PLACEMENT_3D('',#202088,#121941,#121942);
#102899=AXIS2_PLACEMENT_3D('',#202089,#121943,#121944);
#102900=AXIS2_PLACEMENT_3D('',#202090,#121945,#121946);
#102901=AXIS2_PLACEMENT_3D('',#202091,#121947,#121948);
#102902=AXIS2_PLACEMENT_3D('',#202104,#121949,#121950);
#102903=AXIS2_PLACEMENT_3D('',#202123,#121951,#121952);
#102904=AXIS2_PLACEMENT_3D('',#202124,#121953,#121954);
#102905=AXIS2_PLACEMENT_3D('',#202125,#121955,#121956);
#102906=AXIS2_PLACEMENT_3D('',#202126,#121957,#121958);
#102907=AXIS2_PLACEMENT_3D('',#202127,#121959,#121960);
#102908=AXIS2_PLACEMENT_3D('',#202146,#121961,#121962);
#102909=AXIS2_PLACEMENT_3D('',#202159,#121963,#121964);
#102910=AXIS2_PLACEMENT_3D('',#202160,#121965,#121966);
#102911=AXIS2_PLACEMENT_3D('',#202161,#121967,#121968);
#102912=AXIS2_PLACEMENT_3D('',#202162,#121969,#121970);
#102913=AXIS2_PLACEMENT_3D('',#202163,#121971,#121972);
#102914=AXIS2_PLACEMENT_3D('',#202182,#121973,#121974);
#102915=AXIS2_PLACEMENT_3D('',#202183,#121975,#121976);
#102916=AXIS2_PLACEMENT_3D('',#202184,#121977,#121978);
#102917=AXIS2_PLACEMENT_3D('',#202185,#121979,#121980);
#102918=AXIS2_PLACEMENT_3D('',#202186,#121981,#121982);
#102919=AXIS2_PLACEMENT_3D('',#202199,#121983,#121984);
#102920=AXIS2_PLACEMENT_3D('',#202212,#121985,#121986);
#102921=AXIS2_PLACEMENT_3D('',#202213,#121987,#121988);
#102922=AXIS2_PLACEMENT_3D('',#202214,#121989,#121990);
#102923=AXIS2_PLACEMENT_3D('',#202215,#121991,#121992);
#102924=AXIS2_PLACEMENT_3D('',#202216,#121993,#121994);
#102925=AXIS2_PLACEMENT_3D('',#202229,#121995,#121996);
#102926=AXIS2_PLACEMENT_3D('',#202230,#121997,#121998);
#102927=AXIS2_PLACEMENT_3D('',#202231,#121999,#122000);
#102928=AXIS2_PLACEMENT_3D('',#202232,#122001,#122002);
#102929=AXIS2_PLACEMENT_3D('',#202233,#122003,#122004);
#102930=AXIS2_PLACEMENT_3D('',#202246,#122005,#122006);
#102931=AXIS2_PLACEMENT_3D('',#202247,#122007,#122008);
#102932=AXIS2_PLACEMENT_3D('',#202248,#122009,#122010);
#102933=AXIS2_PLACEMENT_3D('',#202249,#122011,#122012);
#102934=AXIS2_PLACEMENT_3D('',#202250,#122013,#122014);
#102935=AXIS2_PLACEMENT_3D('',#202263,#122015,#122016);
#102936=AXIS2_PLACEMENT_3D('',#202276,#122017,#122018);
#102937=AXIS2_PLACEMENT_3D('',#202277,#122019,#122020);
#102938=AXIS2_PLACEMENT_3D('',#202278,#122021,#122022);
#102939=AXIS2_PLACEMENT_3D('',#202279,#122023,#122024);
#102940=AXIS2_PLACEMENT_3D('',#202280,#122025,#122026);
#102941=AXIS2_PLACEMENT_3D('',#202299,#122027,#122028);
#102942=AXIS2_PLACEMENT_3D('',#202300,#122029,#122030);
#102943=AXIS2_PLACEMENT_3D('',#202301,#122031,#122032);
#102944=AXIS2_PLACEMENT_3D('',#202302,#122033,#122034);
#102945=AXIS2_PLACEMENT_3D('',#202303,#122035,#122036);
#102946=AXIS2_PLACEMENT_3D('',#202316,#122037,#122038);
#102947=AXIS2_PLACEMENT_3D('',#202335,#122039,#122040);
#102948=AXIS2_PLACEMENT_3D('',#202336,#122041,#122042);
#102949=AXIS2_PLACEMENT_3D('',#202337,#122043,#122044);
#102950=AXIS2_PLACEMENT_3D('',#202338,#122045,#122046);
#102951=AXIS2_PLACEMENT_3D('',#202339,#122047,#122048);
#102952=AXIS2_PLACEMENT_3D('',#202358,#122049,#122050);
#102953=AXIS2_PLACEMENT_3D('',#202371,#122051,#122052);
#102954=AXIS2_PLACEMENT_3D('',#202372,#122053,#122054);
#102955=AXIS2_PLACEMENT_3D('',#202373,#122055,#122056);
#102956=AXIS2_PLACEMENT_3D('',#202374,#122057,#122058);
#102957=AXIS2_PLACEMENT_3D('',#202375,#122059,#122060);
#102958=AXIS2_PLACEMENT_3D('',#202394,#122061,#122062);
#102959=AXIS2_PLACEMENT_3D('',#202395,#122063,#122064);
#102960=AXIS2_PLACEMENT_3D('',#202396,#122065,#122066);
#102961=AXIS2_PLACEMENT_3D('',#202397,#122067,#122068);
#102962=AXIS2_PLACEMENT_3D('',#202398,#122069,#122070);
#102963=AXIS2_PLACEMENT_3D('',#202411,#122071,#122072);
#102964=AXIS2_PLACEMENT_3D('',#202424,#122073,#122074);
#102965=AXIS2_PLACEMENT_3D('',#202425,#122075,#122076);
#102966=AXIS2_PLACEMENT_3D('',#202426,#122077,#122078);
#102967=AXIS2_PLACEMENT_3D('',#202427,#122079,#122080);
#102968=AXIS2_PLACEMENT_3D('',#202428,#122081,#122082);
#102969=AXIS2_PLACEMENT_3D('',#202441,#122083,#122084);
#102970=AXIS2_PLACEMENT_3D('',#202442,#122085,#122086);
#102971=AXIS2_PLACEMENT_3D('',#202443,#122087,#122088);
#102972=AXIS2_PLACEMENT_3D('',#202444,#122089,#122090);
#102973=AXIS2_PLACEMENT_3D('',#202445,#122091,#122092);
#102974=AXIS2_PLACEMENT_3D('',#202458,#122093,#122094);
#102975=AXIS2_PLACEMENT_3D('',#202459,#122095,#122096);
#102976=AXIS2_PLACEMENT_3D('',#202460,#122097,#122098);
#102977=AXIS2_PLACEMENT_3D('',#202461,#122099,#122100);
#102978=AXIS2_PLACEMENT_3D('',#202462,#122101,#122102);
#102979=AXIS2_PLACEMENT_3D('',#202475,#122103,#122104);
#102980=AXIS2_PLACEMENT_3D('',#202488,#122105,#122106);
#102981=AXIS2_PLACEMENT_3D('',#202489,#122107,#122108);
#102982=AXIS2_PLACEMENT_3D('',#202490,#122109,#122110);
#102983=AXIS2_PLACEMENT_3D('',#202491,#122111,#122112);
#102984=AXIS2_PLACEMENT_3D('',#202492,#122113,#122114);
#102985=AXIS2_PLACEMENT_3D('',#202511,#122115,#122116);
#102986=AXIS2_PLACEMENT_3D('',#202512,#122117,#122118);
#102987=AXIS2_PLACEMENT_3D('',#202513,#122119,#122120);
#102988=AXIS2_PLACEMENT_3D('',#202514,#122121,#122122);
#102989=AXIS2_PLACEMENT_3D('',#202515,#122123,#122124);
#102990=AXIS2_PLACEMENT_3D('',#202528,#122125,#122126);
#102991=AXIS2_PLACEMENT_3D('',#202547,#122127,#122128);
#102992=AXIS2_PLACEMENT_3D('',#202548,#122129,#122130);
#102993=AXIS2_PLACEMENT_3D('',#202549,#122131,#122132);
#102994=AXIS2_PLACEMENT_3D('',#202550,#122133,#122134);
#102995=AXIS2_PLACEMENT_3D('',#202551,#122135,#122136);
#102996=AXIS2_PLACEMENT_3D('',#202570,#122137,#122138);
#102997=AXIS2_PLACEMENT_3D('',#202583,#122139,#122140);
#102998=AXIS2_PLACEMENT_3D('',#202584,#122141,#122142);
#102999=AXIS2_PLACEMENT_3D('',#202585,#122143,#122144);
#103000=AXIS2_PLACEMENT_3D('',#202586,#122145,#122146);
#103001=AXIS2_PLACEMENT_3D('',#202587,#122147,#122148);
#103002=AXIS2_PLACEMENT_3D('',#202606,#122149,#122150);
#103003=AXIS2_PLACEMENT_3D('',#202607,#122151,#122152);
#103004=AXIS2_PLACEMENT_3D('',#202608,#122153,#122154);
#103005=AXIS2_PLACEMENT_3D('',#202609,#122155,#122156);
#103006=AXIS2_PLACEMENT_3D('',#202610,#122157,#122158);
#103007=AXIS2_PLACEMENT_3D('',#202623,#122159,#122160);
#103008=AXIS2_PLACEMENT_3D('',#202636,#122161,#122162);
#103009=AXIS2_PLACEMENT_3D('',#202637,#122163,#122164);
#103010=AXIS2_PLACEMENT_3D('',#202638,#122165,#122166);
#103011=AXIS2_PLACEMENT_3D('',#202639,#122167,#122168);
#103012=AXIS2_PLACEMENT_3D('',#202640,#122169,#122170);
#103013=AXIS2_PLACEMENT_3D('',#202653,#122171,#122172);
#103014=AXIS2_PLACEMENT_3D('',#202654,#122173,#122174);
#103015=AXIS2_PLACEMENT_3D('',#202655,#122175,#122176);
#103016=AXIS2_PLACEMENT_3D('',#202656,#122177,#122178);
#103017=AXIS2_PLACEMENT_3D('',#202657,#122179,#122180);
#103018=AXIS2_PLACEMENT_3D('',#202670,#122181,#122182);
#103019=AXIS2_PLACEMENT_3D('',#202671,#122183,#122184);
#103020=AXIS2_PLACEMENT_3D('',#202672,#122185,#122186);
#103021=AXIS2_PLACEMENT_3D('',#202673,#122187,#122188);
#103022=AXIS2_PLACEMENT_3D('',#202674,#122189,#122190);
#103023=AXIS2_PLACEMENT_3D('',#202687,#122191,#122192);
#103024=AXIS2_PLACEMENT_3D('',#202700,#122193,#122194);
#103025=AXIS2_PLACEMENT_3D('',#202701,#122195,#122196);
#103026=AXIS2_PLACEMENT_3D('',#202702,#122197,#122198);
#103027=AXIS2_PLACEMENT_3D('',#202703,#122199,#122200);
#103028=AXIS2_PLACEMENT_3D('',#202704,#122201,#122202);
#103029=AXIS2_PLACEMENT_3D('',#202723,#122203,#122204);
#103030=AXIS2_PLACEMENT_3D('',#202724,#122205,#122206);
#103031=AXIS2_PLACEMENT_3D('',#202725,#122207,#122208);
#103032=AXIS2_PLACEMENT_3D('',#202726,#122209,#122210);
#103033=AXIS2_PLACEMENT_3D('',#202727,#122211,#122212);
#103034=AXIS2_PLACEMENT_3D('',#202740,#122213,#122214);
#103035=AXIS2_PLACEMENT_3D('',#202759,#122215,#122216);
#103036=AXIS2_PLACEMENT_3D('',#202760,#122217,#122218);
#103037=AXIS2_PLACEMENT_3D('',#202761,#122219,#122220);
#103038=AXIS2_PLACEMENT_3D('',#202762,#122221,#122222);
#103039=AXIS2_PLACEMENT_3D('',#202763,#122223,#122224);
#103040=AXIS2_PLACEMENT_3D('',#202782,#122225,#122226);
#103041=AXIS2_PLACEMENT_3D('',#202795,#122227,#122228);
#103042=AXIS2_PLACEMENT_3D('',#202796,#122229,#122230);
#103043=AXIS2_PLACEMENT_3D('',#202797,#122231,#122232);
#103044=AXIS2_PLACEMENT_3D('',#202798,#122233,#122234);
#103045=AXIS2_PLACEMENT_3D('',#202799,#122235,#122236);
#103046=AXIS2_PLACEMENT_3D('',#202818,#122237,#122238);
#103047=AXIS2_PLACEMENT_3D('',#202819,#122239,#122240);
#103048=AXIS2_PLACEMENT_3D('',#202820,#122241,#122242);
#103049=AXIS2_PLACEMENT_3D('',#202821,#122243,#122244);
#103050=AXIS2_PLACEMENT_3D('',#202822,#122245,#122246);
#103051=AXIS2_PLACEMENT_3D('',#202835,#122247,#122248);
#103052=AXIS2_PLACEMENT_3D('',#202848,#122249,#122250);
#103053=AXIS2_PLACEMENT_3D('',#202849,#122251,#122252);
#103054=AXIS2_PLACEMENT_3D('',#202850,#122253,#122254);
#103055=AXIS2_PLACEMENT_3D('',#202851,#122255,#122256);
#103056=AXIS2_PLACEMENT_3D('',#202852,#122257,#122258);
#103057=AXIS2_PLACEMENT_3D('',#202865,#122259,#122260);
#103058=AXIS2_PLACEMENT_3D('',#202866,#122261,#122262);
#103059=AXIS2_PLACEMENT_3D('',#202867,#122263,#122264);
#103060=AXIS2_PLACEMENT_3D('',#202868,#122265,#122266);
#103061=AXIS2_PLACEMENT_3D('',#202869,#122267,#122268);
#103062=AXIS2_PLACEMENT_3D('',#202882,#122269,#122270);
#103063=AXIS2_PLACEMENT_3D('',#202883,#122271,#122272);
#103064=AXIS2_PLACEMENT_3D('',#202884,#122273,#122274);
#103065=AXIS2_PLACEMENT_3D('',#202885,#122275,#122276);
#103066=AXIS2_PLACEMENT_3D('',#202886,#122277,#122278);
#103067=AXIS2_PLACEMENT_3D('',#202899,#122279,#122280);
#103068=AXIS2_PLACEMENT_3D('',#202912,#122281,#122282);
#103069=AXIS2_PLACEMENT_3D('',#202913,#122283,#122284);
#103070=AXIS2_PLACEMENT_3D('',#202914,#122285,#122286);
#103071=AXIS2_PLACEMENT_3D('',#202915,#122287,#122288);
#103072=AXIS2_PLACEMENT_3D('',#202916,#122289,#122290);
#103073=AXIS2_PLACEMENT_3D('',#202935,#122291,#122292);
#103074=AXIS2_PLACEMENT_3D('',#202936,#122293,#122294);
#103075=AXIS2_PLACEMENT_3D('',#202937,#122295,#122296);
#103076=AXIS2_PLACEMENT_3D('',#202938,#122297,#122298);
#103077=AXIS2_PLACEMENT_3D('',#202939,#122299,#122300);
#103078=AXIS2_PLACEMENT_3D('',#202952,#122301,#122302);
#103079=AXIS2_PLACEMENT_3D('',#202971,#122303,#122304);
#103080=AXIS2_PLACEMENT_3D('',#202972,#122305,#122306);
#103081=AXIS2_PLACEMENT_3D('',#202973,#122307,#122308);
#103082=AXIS2_PLACEMENT_3D('',#202974,#122309,#122310);
#103083=AXIS2_PLACEMENT_3D('',#202975,#122311,#122312);
#103084=AXIS2_PLACEMENT_3D('',#202994,#122313,#122314);
#103085=AXIS2_PLACEMENT_3D('',#203007,#122315,#122316);
#103086=AXIS2_PLACEMENT_3D('',#203008,#122317,#122318);
#103087=AXIS2_PLACEMENT_3D('',#203009,#122319,#122320);
#103088=AXIS2_PLACEMENT_3D('',#203010,#122321,#122322);
#103089=AXIS2_PLACEMENT_3D('',#203011,#122323,#122324);
#103090=AXIS2_PLACEMENT_3D('',#203030,#122325,#122326);
#103091=AXIS2_PLACEMENT_3D('',#203031,#122327,#122328);
#103092=AXIS2_PLACEMENT_3D('',#203032,#122329,#122330);
#103093=AXIS2_PLACEMENT_3D('',#203033,#122331,#122332);
#103094=AXIS2_PLACEMENT_3D('',#203034,#122333,#122334);
#103095=AXIS2_PLACEMENT_3D('',#203047,#122335,#122336);
#103096=AXIS2_PLACEMENT_3D('',#203060,#122337,#122338);
#103097=AXIS2_PLACEMENT_3D('',#203061,#122339,#122340);
#103098=AXIS2_PLACEMENT_3D('',#203062,#122341,#122342);
#103099=AXIS2_PLACEMENT_3D('',#203063,#122343,#122344);
#103100=AXIS2_PLACEMENT_3D('',#203064,#122345,#122346);
#103101=AXIS2_PLACEMENT_3D('',#203077,#122347,#122348);
#103102=AXIS2_PLACEMENT_3D('',#203078,#122349,#122350);
#103103=AXIS2_PLACEMENT_3D('',#203079,#122351,#122352);
#103104=AXIS2_PLACEMENT_3D('',#203080,#122353,#122354);
#103105=AXIS2_PLACEMENT_3D('',#203081,#122355,#122356);
#103106=AXIS2_PLACEMENT_3D('',#203094,#122357,#122358);
#103107=AXIS2_PLACEMENT_3D('',#203095,#122359,#122360);
#103108=AXIS2_PLACEMENT_3D('',#203096,#122361,#122362);
#103109=AXIS2_PLACEMENT_3D('',#203097,#122363,#122364);
#103110=AXIS2_PLACEMENT_3D('',#203098,#122365,#122366);
#103111=AXIS2_PLACEMENT_3D('',#203111,#122367,#122368);
#103112=AXIS2_PLACEMENT_3D('',#203124,#122369,#122370);
#103113=AXIS2_PLACEMENT_3D('',#203125,#122371,#122372);
#103114=AXIS2_PLACEMENT_3D('',#203126,#122373,#122374);
#103115=AXIS2_PLACEMENT_3D('',#203127,#122375,#122376);
#103116=AXIS2_PLACEMENT_3D('',#203128,#122377,#122378);
#103117=AXIS2_PLACEMENT_3D('',#203147,#122379,#122380);
#103118=AXIS2_PLACEMENT_3D('',#203148,#122381,#122382);
#103119=AXIS2_PLACEMENT_3D('',#203149,#122383,#122384);
#103120=AXIS2_PLACEMENT_3D('',#203150,#122385,#122386);
#103121=AXIS2_PLACEMENT_3D('',#203151,#122387,#122388);
#103122=AXIS2_PLACEMENT_3D('',#203164,#122389,#122390);
#103123=AXIS2_PLACEMENT_3D('',#203183,#122391,#122392);
#103124=AXIS2_PLACEMENT_3D('',#203184,#122393,#122394);
#103125=AXIS2_PLACEMENT_3D('',#203185,#122395,#122396);
#103126=AXIS2_PLACEMENT_3D('',#203186,#122397,#122398);
#103127=AXIS2_PLACEMENT_3D('',#203187,#122399,#122400);
#103128=AXIS2_PLACEMENT_3D('',#203206,#122401,#122402);
#103129=AXIS2_PLACEMENT_3D('',#203219,#122403,#122404);
#103130=AXIS2_PLACEMENT_3D('',#203220,#122405,#122406);
#103131=AXIS2_PLACEMENT_3D('',#203221,#122407,#122408);
#103132=AXIS2_PLACEMENT_3D('',#203222,#122409,#122410);
#103133=AXIS2_PLACEMENT_3D('',#203223,#122411,#122412);
#103134=AXIS2_PLACEMENT_3D('',#203242,#122413,#122414);
#103135=AXIS2_PLACEMENT_3D('',#203243,#122415,#122416);
#103136=AXIS2_PLACEMENT_3D('',#203244,#122417,#122418);
#103137=AXIS2_PLACEMENT_3D('',#203245,#122419,#122420);
#103138=AXIS2_PLACEMENT_3D('',#203246,#122421,#122422);
#103139=AXIS2_PLACEMENT_3D('',#203259,#122423,#122424);
#103140=AXIS2_PLACEMENT_3D('',#203272,#122425,#122426);
#103141=AXIS2_PLACEMENT_3D('',#203273,#122427,#122428);
#103142=AXIS2_PLACEMENT_3D('',#203274,#122429,#122430);
#103143=AXIS2_PLACEMENT_3D('',#203275,#122431,#122432);
#103144=AXIS2_PLACEMENT_3D('',#203276,#122433,#122434);
#103145=AXIS2_PLACEMENT_3D('',#203289,#122435,#122436);
#103146=AXIS2_PLACEMENT_3D('',#203290,#122437,#122438);
#103147=AXIS2_PLACEMENT_3D('',#203291,#122439,#122440);
#103148=AXIS2_PLACEMENT_3D('',#203292,#122441,#122442);
#103149=AXIS2_PLACEMENT_3D('',#203293,#122443,#122444);
#103150=AXIS2_PLACEMENT_3D('',#203306,#122445,#122446);
#103151=AXIS2_PLACEMENT_3D('',#203307,#122447,#122448);
#103152=AXIS2_PLACEMENT_3D('',#203308,#122449,#122450);
#103153=AXIS2_PLACEMENT_3D('',#203309,#122451,#122452);
#103154=AXIS2_PLACEMENT_3D('',#203310,#122453,#122454);
#103155=AXIS2_PLACEMENT_3D('',#203323,#122455,#122456);
#103156=AXIS2_PLACEMENT_3D('',#203336,#122457,#122458);
#103157=AXIS2_PLACEMENT_3D('',#203337,#122459,#122460);
#103158=AXIS2_PLACEMENT_3D('',#203338,#122461,#122462);
#103159=AXIS2_PLACEMENT_3D('',#203339,#122463,#122464);
#103160=AXIS2_PLACEMENT_3D('',#203340,#122465,#122466);
#103161=AXIS2_PLACEMENT_3D('',#203359,#122467,#122468);
#103162=AXIS2_PLACEMENT_3D('',#203360,#122469,#122470);
#103163=AXIS2_PLACEMENT_3D('',#203361,#122471,#122472);
#103164=AXIS2_PLACEMENT_3D('',#203362,#122473,#122474);
#103165=AXIS2_PLACEMENT_3D('',#203363,#122475,#122476);
#103166=AXIS2_PLACEMENT_3D('',#203376,#122477,#122478);
#103167=AXIS2_PLACEMENT_3D('',#203395,#122479,#122480);
#103168=AXIS2_PLACEMENT_3D('',#203396,#122481,#122482);
#103169=AXIS2_PLACEMENT_3D('',#203397,#122483,#122484);
#103170=AXIS2_PLACEMENT_3D('',#203398,#122485,#122486);
#103171=AXIS2_PLACEMENT_3D('',#203399,#122487,#122488);
#103172=AXIS2_PLACEMENT_3D('',#203418,#122489,#122490);
#103173=AXIS2_PLACEMENT_3D('',#203431,#122491,#122492);
#103174=AXIS2_PLACEMENT_3D('',#203432,#122493,#122494);
#103175=AXIS2_PLACEMENT_3D('',#203433,#122495,#122496);
#103176=AXIS2_PLACEMENT_3D('',#203434,#122497,#122498);
#103177=AXIS2_PLACEMENT_3D('',#203435,#122499,#122500);
#103178=AXIS2_PLACEMENT_3D('',#203454,#122501,#122502);
#103179=AXIS2_PLACEMENT_3D('',#203455,#122503,#122504);
#103180=AXIS2_PLACEMENT_3D('',#203456,#122505,#122506);
#103181=AXIS2_PLACEMENT_3D('',#203457,#122507,#122508);
#103182=AXIS2_PLACEMENT_3D('',#203458,#122509,#122510);
#103183=AXIS2_PLACEMENT_3D('',#203471,#122511,#122512);
#103184=AXIS2_PLACEMENT_3D('',#203484,#122513,#122514);
#103185=AXIS2_PLACEMENT_3D('',#203485,#122515,#122516);
#103186=AXIS2_PLACEMENT_3D('',#203486,#122517,#122518);
#103187=AXIS2_PLACEMENT_3D('',#203487,#122519,#122520);
#103188=AXIS2_PLACEMENT_3D('',#203488,#122521,#122522);
#103189=AXIS2_PLACEMENT_3D('',#203501,#122523,#122524);
#103190=AXIS2_PLACEMENT_3D('',#203502,#122525,#122526);
#103191=AXIS2_PLACEMENT_3D('',#203503,#122527,#122528);
#103192=AXIS2_PLACEMENT_3D('',#203504,#122529,#122530);
#103193=AXIS2_PLACEMENT_3D('',#203505,#122531,#122532);
#103194=AXIS2_PLACEMENT_3D('',#203518,#122533,#122534);
#103195=AXIS2_PLACEMENT_3D('',#203519,#122535,#122536);
#103196=AXIS2_PLACEMENT_3D('',#203520,#122537,#122538);
#103197=AXIS2_PLACEMENT_3D('',#203521,#122539,#122540);
#103198=AXIS2_PLACEMENT_3D('',#203522,#122541,#122542);
#103199=AXIS2_PLACEMENT_3D('',#203535,#122543,#122544);
#103200=AXIS2_PLACEMENT_3D('',#203548,#122545,#122546);
#103201=AXIS2_PLACEMENT_3D('',#203549,#122547,#122548);
#103202=AXIS2_PLACEMENT_3D('',#203550,#122549,#122550);
#103203=AXIS2_PLACEMENT_3D('',#203551,#122551,#122552);
#103204=AXIS2_PLACEMENT_3D('',#203552,#122553,#122554);
#103205=AXIS2_PLACEMENT_3D('',#203571,#122555,#122556);
#103206=AXIS2_PLACEMENT_3D('',#203572,#122557,#122558);
#103207=AXIS2_PLACEMENT_3D('',#203573,#122559,#122560);
#103208=AXIS2_PLACEMENT_3D('',#203574,#122561,#122562);
#103209=AXIS2_PLACEMENT_3D('',#203575,#122563,#122564);
#103210=AXIS2_PLACEMENT_3D('',#203588,#122565,#122566);
#103211=AXIS2_PLACEMENT_3D('',#203607,#122567,#122568);
#103212=AXIS2_PLACEMENT_3D('',#203608,#122569,#122570);
#103213=AXIS2_PLACEMENT_3D('',#203609,#122571,#122572);
#103214=AXIS2_PLACEMENT_3D('',#203610,#122573,#122574);
#103215=AXIS2_PLACEMENT_3D('',#203611,#122575,#122576);
#103216=AXIS2_PLACEMENT_3D('',#203630,#122577,#122578);
#103217=AXIS2_PLACEMENT_3D('',#203643,#122579,#122580);
#103218=AXIS2_PLACEMENT_3D('',#203644,#122581,#122582);
#103219=AXIS2_PLACEMENT_3D('',#203645,#122583,#122584);
#103220=AXIS2_PLACEMENT_3D('',#203646,#122585,#122586);
#103221=AXIS2_PLACEMENT_3D('',#203647,#122587,#122588);
#103222=AXIS2_PLACEMENT_3D('',#203666,#122589,#122590);
#103223=AXIS2_PLACEMENT_3D('',#203667,#122591,#122592);
#103224=AXIS2_PLACEMENT_3D('',#203668,#122593,#122594);
#103225=AXIS2_PLACEMENT_3D('',#203669,#122595,#122596);
#103226=AXIS2_PLACEMENT_3D('',#203670,#122597,#122598);
#103227=AXIS2_PLACEMENT_3D('',#203683,#122599,#122600);
#103228=AXIS2_PLACEMENT_3D('',#203696,#122601,#122602);
#103229=AXIS2_PLACEMENT_3D('',#203697,#122603,#122604);
#103230=AXIS2_PLACEMENT_3D('',#203698,#122605,#122606);
#103231=AXIS2_PLACEMENT_3D('',#203699,#122607,#122608);
#103232=AXIS2_PLACEMENT_3D('',#203700,#122609,#122610);
#103233=AXIS2_PLACEMENT_3D('',#203713,#122611,#122612);
#103234=AXIS2_PLACEMENT_3D('',#203714,#122613,#122614);
#103235=AXIS2_PLACEMENT_3D('',#203715,#122615,#122616);
#103236=AXIS2_PLACEMENT_3D('',#203716,#122617,#122618);
#103237=AXIS2_PLACEMENT_3D('',#203717,#122619,#122620);
#103238=AXIS2_PLACEMENT_3D('',#203730,#122621,#122622);
#103239=AXIS2_PLACEMENT_3D('',#203731,#122623,#122624);
#103240=AXIS2_PLACEMENT_3D('',#203732,#122625,#122626);
#103241=AXIS2_PLACEMENT_3D('',#203733,#122627,#122628);
#103242=AXIS2_PLACEMENT_3D('',#203734,#122629,#122630);
#103243=AXIS2_PLACEMENT_3D('',#203747,#122631,#122632);
#103244=AXIS2_PLACEMENT_3D('',#203760,#122633,#122634);
#103245=AXIS2_PLACEMENT_3D('',#203761,#122635,#122636);
#103246=AXIS2_PLACEMENT_3D('',#203762,#122637,#122638);
#103247=AXIS2_PLACEMENT_3D('',#203763,#122639,#122640);
#103248=AXIS2_PLACEMENT_3D('',#203764,#122641,#122642);
#103249=AXIS2_PLACEMENT_3D('',#203783,#122643,#122644);
#103250=AXIS2_PLACEMENT_3D('',#203784,#122645,#122646);
#103251=AXIS2_PLACEMENT_3D('',#203785,#122647,#122648);
#103252=AXIS2_PLACEMENT_3D('',#203786,#122649,#122650);
#103253=AXIS2_PLACEMENT_3D('',#203787,#122651,#122652);
#103254=AXIS2_PLACEMENT_3D('',#203800,#122653,#122654);
#103255=AXIS2_PLACEMENT_3D('',#203819,#122655,#122656);
#103256=AXIS2_PLACEMENT_3D('',#203820,#122657,#122658);
#103257=AXIS2_PLACEMENT_3D('',#203821,#122659,#122660);
#103258=AXIS2_PLACEMENT_3D('',#203822,#122661,#122662);
#103259=AXIS2_PLACEMENT_3D('',#203823,#122663,#122664);
#103260=AXIS2_PLACEMENT_3D('',#203842,#122665,#122666);
#103261=AXIS2_PLACEMENT_3D('',#203855,#122667,#122668);
#103262=AXIS2_PLACEMENT_3D('',#203856,#122669,#122670);
#103263=AXIS2_PLACEMENT_3D('',#203857,#122671,#122672);
#103264=AXIS2_PLACEMENT_3D('',#203858,#122673,#122674);
#103265=AXIS2_PLACEMENT_3D('',#203859,#122675,#122676);
#103266=AXIS2_PLACEMENT_3D('',#203878,#122677,#122678);
#103267=AXIS2_PLACEMENT_3D('',#203879,#122679,#122680);
#103268=AXIS2_PLACEMENT_3D('',#203880,#122681,#122682);
#103269=AXIS2_PLACEMENT_3D('',#203881,#122683,#122684);
#103270=AXIS2_PLACEMENT_3D('',#203882,#122685,#122686);
#103271=AXIS2_PLACEMENT_3D('',#203895,#122687,#122688);
#103272=AXIS2_PLACEMENT_3D('',#203908,#122689,#122690);
#103273=AXIS2_PLACEMENT_3D('',#203909,#122691,#122692);
#103274=AXIS2_PLACEMENT_3D('',#203910,#122693,#122694);
#103275=AXIS2_PLACEMENT_3D('',#203911,#122695,#122696);
#103276=AXIS2_PLACEMENT_3D('',#203912,#122697,#122698);
#103277=AXIS2_PLACEMENT_3D('',#203925,#122699,#122700);
#103278=AXIS2_PLACEMENT_3D('',#203926,#122701,#122702);
#103279=AXIS2_PLACEMENT_3D('',#203927,#122703,#122704);
#103280=AXIS2_PLACEMENT_3D('',#203928,#122705,#122706);
#103281=AXIS2_PLACEMENT_3D('',#203929,#122707,#122708);
#103282=AXIS2_PLACEMENT_3D('',#203942,#122709,#122710);
#103283=AXIS2_PLACEMENT_3D('',#203943,#122711,#122712);
#103284=AXIS2_PLACEMENT_3D('',#203944,#122713,#122714);
#103285=AXIS2_PLACEMENT_3D('',#203945,#122715,#122716);
#103286=AXIS2_PLACEMENT_3D('',#203946,#122717,#122718);
#103287=AXIS2_PLACEMENT_3D('',#203959,#122719,#122720);
#103288=AXIS2_PLACEMENT_3D('',#203972,#122721,#122722);
#103289=AXIS2_PLACEMENT_3D('',#203973,#122723,#122724);
#103290=AXIS2_PLACEMENT_3D('',#203974,#122725,#122726);
#103291=AXIS2_PLACEMENT_3D('',#203975,#122727,#122728);
#103292=AXIS2_PLACEMENT_3D('',#203976,#122729,#122730);
#103293=AXIS2_PLACEMENT_3D('',#203995,#122731,#122732);
#103294=AXIS2_PLACEMENT_3D('',#203996,#122733,#122734);
#103295=AXIS2_PLACEMENT_3D('',#203997,#122735,#122736);
#103296=AXIS2_PLACEMENT_3D('',#203998,#122737,#122738);
#103297=AXIS2_PLACEMENT_3D('',#203999,#122739,#122740);
#103298=AXIS2_PLACEMENT_3D('',#204012,#122741,#122742);
#103299=AXIS2_PLACEMENT_3D('',#204031,#122743,#122744);
#103300=AXIS2_PLACEMENT_3D('',#204032,#122745,#122746);
#103301=AXIS2_PLACEMENT_3D('',#204033,#122747,#122748);
#103302=AXIS2_PLACEMENT_3D('',#204034,#122749,#122750);
#103303=AXIS2_PLACEMENT_3D('',#204035,#122751,#122752);
#103304=AXIS2_PLACEMENT_3D('',#204054,#122753,#122754);
#103305=AXIS2_PLACEMENT_3D('',#204067,#122755,#122756);
#103306=AXIS2_PLACEMENT_3D('',#204068,#122757,#122758);
#103307=AXIS2_PLACEMENT_3D('',#204069,#122759,#122760);
#103308=AXIS2_PLACEMENT_3D('',#204070,#122761,#122762);
#103309=AXIS2_PLACEMENT_3D('',#204071,#122763,#122764);
#103310=AXIS2_PLACEMENT_3D('',#204090,#122765,#122766);
#103311=AXIS2_PLACEMENT_3D('',#204091,#122767,#122768);
#103312=AXIS2_PLACEMENT_3D('',#204092,#122769,#122770);
#103313=AXIS2_PLACEMENT_3D('',#204093,#122771,#122772);
#103314=AXIS2_PLACEMENT_3D('',#204094,#122773,#122774);
#103315=AXIS2_PLACEMENT_3D('',#204107,#122775,#122776);
#103316=AXIS2_PLACEMENT_3D('',#204120,#122777,#122778);
#103317=AXIS2_PLACEMENT_3D('',#204121,#122779,#122780);
#103318=AXIS2_PLACEMENT_3D('',#204122,#122781,#122782);
#103319=AXIS2_PLACEMENT_3D('',#204123,#122783,#122784);
#103320=AXIS2_PLACEMENT_3D('',#204124,#122785,#122786);
#103321=AXIS2_PLACEMENT_3D('',#204137,#122787,#122788);
#103322=AXIS2_PLACEMENT_3D('',#204138,#122789,#122790);
#103323=AXIS2_PLACEMENT_3D('',#204139,#122791,#122792);
#103324=AXIS2_PLACEMENT_3D('',#204140,#122793,#122794);
#103325=AXIS2_PLACEMENT_3D('',#204141,#122795,#122796);
#103326=AXIS2_PLACEMENT_3D('',#204154,#122797,#122798);
#103327=AXIS2_PLACEMENT_3D('',#204155,#122799,#122800);
#103328=AXIS2_PLACEMENT_3D('',#204156,#122801,#122802);
#103329=AXIS2_PLACEMENT_3D('',#204157,#122803,#122804);
#103330=AXIS2_PLACEMENT_3D('',#204158,#122805,#122806);
#103331=AXIS2_PLACEMENT_3D('',#204171,#122807,#122808);
#103332=AXIS2_PLACEMENT_3D('',#204184,#122809,#122810);
#103333=AXIS2_PLACEMENT_3D('',#204185,#122811,#122812);
#103334=AXIS2_PLACEMENT_3D('',#204186,#122813,#122814);
#103335=AXIS2_PLACEMENT_3D('',#204187,#122815,#122816);
#103336=AXIS2_PLACEMENT_3D('',#204188,#122817,#122818);
#103337=AXIS2_PLACEMENT_3D('',#204207,#122819,#122820);
#103338=AXIS2_PLACEMENT_3D('',#204208,#122821,#122822);
#103339=AXIS2_PLACEMENT_3D('',#204221,#122823,#122824);
#103340=AXIS2_PLACEMENT_3D('',#204240,#122825,#122826);
#103341=AXIS2_PLACEMENT_3D('',#204241,#122827,#122828);
#103342=AXIS2_PLACEMENT_3D('',#204242,#122829,#122830);
#103343=AXIS2_PLACEMENT_3D('',#204243,#122831,#122832);
#103344=AXIS2_PLACEMENT_3D('',#204244,#122833,#122834);
#103345=AXIS2_PLACEMENT_3D('',#204275,#122835,#122836);
#103346=AXIS2_PLACEMENT_3D('',#204276,#122837,#122838);
#103347=AXIS2_PLACEMENT_3D('',#204277,#122839,#122840);
#103348=AXIS2_PLACEMENT_3D('',#204296,#122841,#122842);
#103349=AXIS2_PLACEMENT_3D('',#204297,#122843,#122844);
#103350=AXIS2_PLACEMENT_3D('',#204298,#122845,#122846);
#103351=AXIS2_PLACEMENT_3D('',#204299,#122847,#122848);
#103352=AXIS2_PLACEMENT_3D('',#204300,#122849,#122850);
#103353=AXIS2_PLACEMENT_3D('',#204313,#122851,#122852);
#103354=AXIS2_PLACEMENT_3D('',#204326,#122853,#122854);
#103355=AXIS2_PLACEMENT_3D('',#204327,#122855,#122856);
#103356=AXIS2_PLACEMENT_3D('',#204328,#122857,#122858);
#103357=AXIS2_PLACEMENT_3D('',#204329,#122859,#122860);
#103358=AXIS2_PLACEMENT_3D('',#204330,#122861,#122862);
#103359=AXIS2_PLACEMENT_3D('',#204343,#122863,#122864);
#103360=AXIS2_PLACEMENT_3D('',#204344,#122865,#122866);
#103361=AXIS2_PLACEMENT_3D('',#204345,#122867,#122868);
#103362=AXIS2_PLACEMENT_3D('',#204346,#122869,#122870);
#103363=AXIS2_PLACEMENT_3D('',#204347,#122871,#122872);
#103364=AXIS2_PLACEMENT_3D('',#204360,#122873,#122874);
#103365=AXIS2_PLACEMENT_3D('',#204361,#122875,#122876);
#103366=AXIS2_PLACEMENT_3D('',#204362,#122877,#122878);
#103367=AXIS2_PLACEMENT_3D('',#204363,#122879,#122880);
#103368=AXIS2_PLACEMENT_3D('',#204364,#122881,#122882);
#103369=AXIS2_PLACEMENT_3D('',#204377,#122883,#122884);
#103370=AXIS2_PLACEMENT_3D('',#204390,#122885,#122886);
#103371=AXIS2_PLACEMENT_3D('',#204391,#122887,#122888);
#103372=AXIS2_PLACEMENT_3D('',#204392,#122889,#122890);
#103373=AXIS2_PLACEMENT_3D('',#204393,#122891,#122892);
#103374=AXIS2_PLACEMENT_3D('',#204394,#122893,#122894);
#103375=AXIS2_PLACEMENT_3D('',#204413,#122895,#122896);
#103376=AXIS2_PLACEMENT_3D('',#204414,#122897,#122898);
#103377=AXIS2_PLACEMENT_3D('',#204415,#122899,#122900);
#103378=AXIS2_PLACEMENT_3D('',#204416,#122901,#122902);
#103379=AXIS2_PLACEMENT_3D('',#204417,#122903,#122904);
#103380=AXIS2_PLACEMENT_3D('',#204430,#122905,#122906);
#103381=AXIS2_PLACEMENT_3D('',#204449,#122907,#122908);
#103382=AXIS2_PLACEMENT_3D('',#204450,#122909,#122910);
#103383=AXIS2_PLACEMENT_3D('',#204451,#122911,#122912);
#103384=AXIS2_PLACEMENT_3D('',#204452,#122913,#122914);
#103385=AXIS2_PLACEMENT_3D('',#204453,#122915,#122916);
#103386=AXIS2_PLACEMENT_3D('',#204472,#122917,#122918);
#103387=AXIS2_PLACEMENT_3D('',#204485,#122919,#122920);
#103388=AXIS2_PLACEMENT_3D('',#204486,#122921,#122922);
#103389=AXIS2_PLACEMENT_3D('',#204487,#122923,#122924);
#103390=AXIS2_PLACEMENT_3D('',#204488,#122925,#122926);
#103391=AXIS2_PLACEMENT_3D('',#204489,#122927,#122928);
#103392=AXIS2_PLACEMENT_3D('',#204508,#122929,#122930);
#103393=AXIS2_PLACEMENT_3D('',#204509,#122931,#122932);
#103394=AXIS2_PLACEMENT_3D('',#204510,#122933,#122934);
#103395=AXIS2_PLACEMENT_3D('',#204511,#122935,#122936);
#103396=AXIS2_PLACEMENT_3D('',#204512,#122937,#122938);
#103397=AXIS2_PLACEMENT_3D('',#204525,#122939,#122940);
#103398=AXIS2_PLACEMENT_3D('',#204538,#122941,#122942);
#103399=AXIS2_PLACEMENT_3D('',#204539,#122943,#122944);
#103400=AXIS2_PLACEMENT_3D('',#204540,#122945,#122946);
#103401=AXIS2_PLACEMENT_3D('',#204541,#122947,#122948);
#103402=AXIS2_PLACEMENT_3D('',#204542,#122949,#122950);
#103403=AXIS2_PLACEMENT_3D('',#204555,#122951,#122952);
#103404=AXIS2_PLACEMENT_3D('',#204556,#122953,#122954);
#103405=AXIS2_PLACEMENT_3D('',#204557,#122955,#122956);
#103406=AXIS2_PLACEMENT_3D('',#204558,#122957,#122958);
#103407=AXIS2_PLACEMENT_3D('',#204559,#122959,#122960);
#103408=AXIS2_PLACEMENT_3D('',#204572,#122961,#122962);
#103409=AXIS2_PLACEMENT_3D('',#204573,#122963,#122964);
#103410=AXIS2_PLACEMENT_3D('',#204574,#122965,#122966);
#103411=AXIS2_PLACEMENT_3D('',#204575,#122967,#122968);
#103412=AXIS2_PLACEMENT_3D('',#204576,#122969,#122970);
#103413=AXIS2_PLACEMENT_3D('',#204589,#122971,#122972);
#103414=AXIS2_PLACEMENT_3D('',#204602,#122973,#122974);
#103415=AXIS2_PLACEMENT_3D('',#204603,#122975,#122976);
#103416=AXIS2_PLACEMENT_3D('',#204604,#122977,#122978);
#103417=AXIS2_PLACEMENT_3D('',#204605,#122979,#122980);
#103418=AXIS2_PLACEMENT_3D('',#204606,#122981,#122982);
#103419=AXIS2_PLACEMENT_3D('',#204625,#122983,#122984);
#103420=AXIS2_PLACEMENT_3D('',#204626,#122985,#122986);
#103421=AXIS2_PLACEMENT_3D('',#204627,#122987,#122988);
#103422=AXIS2_PLACEMENT_3D('',#204628,#122989,#122990);
#103423=AXIS2_PLACEMENT_3D('',#204629,#122991,#122992);
#103424=AXIS2_PLACEMENT_3D('',#204642,#122993,#122994);
#103425=AXIS2_PLACEMENT_3D('',#204661,#122995,#122996);
#103426=AXIS2_PLACEMENT_3D('',#204662,#122997,#122998);
#103427=AXIS2_PLACEMENT_3D('',#204663,#122999,#123000);
#103428=AXIS2_PLACEMENT_3D('',#204664,#123001,#123002);
#103429=AXIS2_PLACEMENT_3D('',#204665,#123003,#123004);
#103430=AXIS2_PLACEMENT_3D('',#204684,#123005,#123006);
#103431=AXIS2_PLACEMENT_3D('',#204697,#123007,#123008);
#103432=AXIS2_PLACEMENT_3D('',#204698,#123009,#123010);
#103433=AXIS2_PLACEMENT_3D('',#204699,#123011,#123012);
#103434=AXIS2_PLACEMENT_3D('',#204700,#123013,#123014);
#103435=AXIS2_PLACEMENT_3D('',#204701,#123015,#123016);
#103436=AXIS2_PLACEMENT_3D('',#204720,#123017,#123018);
#103437=AXIS2_PLACEMENT_3D('',#204721,#123019,#123020);
#103438=AXIS2_PLACEMENT_3D('',#204722,#123021,#123022);
#103439=AXIS2_PLACEMENT_3D('',#204723,#123023,#123024);
#103440=AXIS2_PLACEMENT_3D('',#204724,#123025,#123026);
#103441=AXIS2_PLACEMENT_3D('',#204737,#123027,#123028);
#103442=AXIS2_PLACEMENT_3D('',#204750,#123029,#123030);
#103443=AXIS2_PLACEMENT_3D('',#204751,#123031,#123032);
#103444=AXIS2_PLACEMENT_3D('',#204752,#123033,#123034);
#103445=AXIS2_PLACEMENT_3D('',#204753,#123035,#123036);
#103446=AXIS2_PLACEMENT_3D('',#204754,#123037,#123038);
#103447=AXIS2_PLACEMENT_3D('',#204767,#123039,#123040);
#103448=AXIS2_PLACEMENT_3D('',#204768,#123041,#123042);
#103449=AXIS2_PLACEMENT_3D('',#204769,#123043,#123044);
#103450=AXIS2_PLACEMENT_3D('',#204770,#123045,#123046);
#103451=AXIS2_PLACEMENT_3D('',#204771,#123047,#123048);
#103452=AXIS2_PLACEMENT_3D('',#204784,#123049,#123050);
#103453=AXIS2_PLACEMENT_3D('',#204785,#123051,#123052);
#103454=AXIS2_PLACEMENT_3D('',#204786,#123053,#123054);
#103455=AXIS2_PLACEMENT_3D('',#204787,#123055,#123056);
#103456=AXIS2_PLACEMENT_3D('',#204788,#123057,#123058);
#103457=AXIS2_PLACEMENT_3D('',#204801,#123059,#123060);
#103458=AXIS2_PLACEMENT_3D('',#204814,#123061,#123062);
#103459=AXIS2_PLACEMENT_3D('',#204815,#123063,#123064);
#103460=AXIS2_PLACEMENT_3D('',#204816,#123065,#123066);
#103461=AXIS2_PLACEMENT_3D('',#204817,#123067,#123068);
#103462=AXIS2_PLACEMENT_3D('',#204818,#123069,#123070);
#103463=AXIS2_PLACEMENT_3D('',#204837,#123071,#123072);
#103464=AXIS2_PLACEMENT_3D('',#204838,#123073,#123074);
#103465=AXIS2_PLACEMENT_3D('',#204839,#123075,#123076);
#103466=AXIS2_PLACEMENT_3D('',#204840,#123077,#123078);
#103467=AXIS2_PLACEMENT_3D('',#204841,#123079,#123080);
#103468=AXIS2_PLACEMENT_3D('',#204854,#123081,#123082);
#103469=AXIS2_PLACEMENT_3D('',#204873,#123083,#123084);
#103470=AXIS2_PLACEMENT_3D('',#204874,#123085,#123086);
#103471=AXIS2_PLACEMENT_3D('',#204875,#123087,#123088);
#103472=AXIS2_PLACEMENT_3D('',#204876,#123089,#123090);
#103473=AXIS2_PLACEMENT_3D('',#204877,#123091,#123092);
#103474=AXIS2_PLACEMENT_3D('',#204896,#123093,#123094);
#103475=AXIS2_PLACEMENT_3D('',#204909,#123095,#123096);
#103476=AXIS2_PLACEMENT_3D('',#204910,#123097,#123098);
#103477=AXIS2_PLACEMENT_3D('',#204911,#123099,#123100);
#103478=AXIS2_PLACEMENT_3D('',#204912,#123101,#123102);
#103479=AXIS2_PLACEMENT_3D('',#204913,#123103,#123104);
#103480=AXIS2_PLACEMENT_3D('',#204932,#123105,#123106);
#103481=AXIS2_PLACEMENT_3D('',#204933,#123107,#123108);
#103482=AXIS2_PLACEMENT_3D('',#204934,#123109,#123110);
#103483=AXIS2_PLACEMENT_3D('',#204935,#123111,#123112);
#103484=AXIS2_PLACEMENT_3D('',#204936,#123113,#123114);
#103485=AXIS2_PLACEMENT_3D('',#204949,#123115,#123116);
#103486=AXIS2_PLACEMENT_3D('',#204962,#123117,#123118);
#103487=AXIS2_PLACEMENT_3D('',#204963,#123119,#123120);
#103488=AXIS2_PLACEMENT_3D('',#204964,#123121,#123122);
#103489=AXIS2_PLACEMENT_3D('',#204965,#123123,#123124);
#103490=AXIS2_PLACEMENT_3D('',#204966,#123125,#123126);
#103491=AXIS2_PLACEMENT_3D('',#204979,#123127,#123128);
#103492=AXIS2_PLACEMENT_3D('',#204980,#123129,#123130);
#103493=AXIS2_PLACEMENT_3D('',#204981,#123131,#123132);
#103494=AXIS2_PLACEMENT_3D('',#204982,#123133,#123134);
#103495=AXIS2_PLACEMENT_3D('',#204983,#123135,#123136);
#103496=AXIS2_PLACEMENT_3D('',#204996,#123137,#123138);
#103497=AXIS2_PLACEMENT_3D('',#204997,#123139,#123140);
#103498=AXIS2_PLACEMENT_3D('',#204998,#123141,#123142);
#103499=AXIS2_PLACEMENT_3D('',#204999,#123143,#123144);
#103500=AXIS2_PLACEMENT_3D('',#205000,#123145,#123146);
#103501=AXIS2_PLACEMENT_3D('',#205013,#123147,#123148);
#103502=AXIS2_PLACEMENT_3D('',#205026,#123149,#123150);
#103503=AXIS2_PLACEMENT_3D('',#205027,#123151,#123152);
#103504=AXIS2_PLACEMENT_3D('',#205028,#123153,#123154);
#103505=AXIS2_PLACEMENT_3D('',#205029,#123155,#123156);
#103506=AXIS2_PLACEMENT_3D('',#205030,#123157,#123158);
#103507=AXIS2_PLACEMENT_3D('',#205049,#123159,#123160);
#103508=AXIS2_PLACEMENT_3D('',#205050,#123161,#123162);
#103509=AXIS2_PLACEMENT_3D('',#205051,#123163,#123164);
#103510=AXIS2_PLACEMENT_3D('',#205052,#123165,#123166);
#103511=AXIS2_PLACEMENT_3D('',#205053,#123167,#123168);
#103512=AXIS2_PLACEMENT_3D('',#205066,#123169,#123170);
#103513=AXIS2_PLACEMENT_3D('',#205085,#123171,#123172);
#103514=AXIS2_PLACEMENT_3D('',#205086,#123173,#123174);
#103515=AXIS2_PLACEMENT_3D('',#205087,#123175,#123176);
#103516=AXIS2_PLACEMENT_3D('',#205088,#123177,#123178);
#103517=AXIS2_PLACEMENT_3D('',#205089,#123179,#123180);
#103518=AXIS2_PLACEMENT_3D('',#205108,#123181,#123182);
#103519=AXIS2_PLACEMENT_3D('',#205121,#123183,#123184);
#103520=AXIS2_PLACEMENT_3D('',#205122,#123185,#123186);
#103521=AXIS2_PLACEMENT_3D('',#205123,#123187,#123188);
#103522=AXIS2_PLACEMENT_3D('',#205124,#123189,#123190);
#103523=AXIS2_PLACEMENT_3D('',#205125,#123191,#123192);
#103524=AXIS2_PLACEMENT_3D('',#205144,#123193,#123194);
#103525=AXIS2_PLACEMENT_3D('',#205145,#123195,#123196);
#103526=AXIS2_PLACEMENT_3D('',#205146,#123197,#123198);
#103527=AXIS2_PLACEMENT_3D('',#205147,#123199,#123200);
#103528=AXIS2_PLACEMENT_3D('',#205148,#123201,#123202);
#103529=AXIS2_PLACEMENT_3D('',#205161,#123203,#123204);
#103530=AXIS2_PLACEMENT_3D('',#205174,#123205,#123206);
#103531=AXIS2_PLACEMENT_3D('',#205175,#123207,#123208);
#103532=AXIS2_PLACEMENT_3D('',#205176,#123209,#123210);
#103533=AXIS2_PLACEMENT_3D('',#205177,#123211,#123212);
#103534=AXIS2_PLACEMENT_3D('',#205178,#123213,#123214);
#103535=AXIS2_PLACEMENT_3D('',#205191,#123215,#123216);
#103536=AXIS2_PLACEMENT_3D('',#205192,#123217,#123218);
#103537=AXIS2_PLACEMENT_3D('',#205193,#123219,#123220);
#103538=AXIS2_PLACEMENT_3D('',#205194,#123221,#123222);
#103539=AXIS2_PLACEMENT_3D('',#205195,#123223,#123224);
#103540=AXIS2_PLACEMENT_3D('',#205208,#123225,#123226);
#103541=AXIS2_PLACEMENT_3D('',#205209,#123227,#123228);
#103542=AXIS2_PLACEMENT_3D('',#205210,#123229,#123230);
#103543=AXIS2_PLACEMENT_3D('',#205211,#123231,#123232);
#103544=AXIS2_PLACEMENT_3D('',#205212,#123233,#123234);
#103545=AXIS2_PLACEMENT_3D('',#205225,#123235,#123236);
#103546=AXIS2_PLACEMENT_3D('',#205238,#123237,#123238);
#103547=AXIS2_PLACEMENT_3D('',#205239,#123239,#123240);
#103548=AXIS2_PLACEMENT_3D('',#205240,#123241,#123242);
#103549=AXIS2_PLACEMENT_3D('',#205241,#123243,#123244);
#103550=AXIS2_PLACEMENT_3D('',#205242,#123245,#123246);
#103551=AXIS2_PLACEMENT_3D('',#205261,#123247,#123248);
#103552=AXIS2_PLACEMENT_3D('',#205262,#123249,#123250);
#103553=AXIS2_PLACEMENT_3D('',#205263,#123251,#123252);
#103554=AXIS2_PLACEMENT_3D('',#205264,#123253,#123254);
#103555=AXIS2_PLACEMENT_3D('',#205265,#123255,#123256);
#103556=AXIS2_PLACEMENT_3D('',#205278,#123257,#123258);
#103557=AXIS2_PLACEMENT_3D('',#205297,#123259,#123260);
#103558=AXIS2_PLACEMENT_3D('',#205298,#123261,#123262);
#103559=AXIS2_PLACEMENT_3D('',#205299,#123263,#123264);
#103560=AXIS2_PLACEMENT_3D('',#205300,#123265,#123266);
#103561=AXIS2_PLACEMENT_3D('',#205301,#123267,#123268);
#103562=AXIS2_PLACEMENT_3D('',#205320,#123269,#123270);
#103563=AXIS2_PLACEMENT_3D('',#205333,#123271,#123272);
#103564=AXIS2_PLACEMENT_3D('',#205334,#123273,#123274);
#103565=AXIS2_PLACEMENT_3D('',#205335,#123275,#123276);
#103566=AXIS2_PLACEMENT_3D('',#205336,#123277,#123278);
#103567=AXIS2_PLACEMENT_3D('',#205337,#123279,#123280);
#103568=AXIS2_PLACEMENT_3D('',#205356,#123281,#123282);
#103569=AXIS2_PLACEMENT_3D('',#205357,#123283,#123284);
#103570=AXIS2_PLACEMENT_3D('',#205358,#123285,#123286);
#103571=AXIS2_PLACEMENT_3D('',#205359,#123287,#123288);
#103572=AXIS2_PLACEMENT_3D('',#205360,#123289,#123290);
#103573=AXIS2_PLACEMENT_3D('',#205373,#123291,#123292);
#103574=AXIS2_PLACEMENT_3D('',#205386,#123293,#123294);
#103575=AXIS2_PLACEMENT_3D('',#205387,#123295,#123296);
#103576=AXIS2_PLACEMENT_3D('',#205388,#123297,#123298);
#103577=AXIS2_PLACEMENT_3D('',#205389,#123299,#123300);
#103578=AXIS2_PLACEMENT_3D('',#205390,#123301,#123302);
#103579=AXIS2_PLACEMENT_3D('',#205403,#123303,#123304);
#103580=AXIS2_PLACEMENT_3D('',#205404,#123305,#123306);
#103581=AXIS2_PLACEMENT_3D('',#205405,#123307,#123308);
#103582=AXIS2_PLACEMENT_3D('',#205406,#123309,#123310);
#103583=AXIS2_PLACEMENT_3D('',#205407,#123311,#123312);
#103584=AXIS2_PLACEMENT_3D('',#205420,#123313,#123314);
#103585=AXIS2_PLACEMENT_3D('',#205421,#123315,#123316);
#103586=AXIS2_PLACEMENT_3D('',#205422,#123317,#123318);
#103587=AXIS2_PLACEMENT_3D('',#205423,#123319,#123320);
#103588=AXIS2_PLACEMENT_3D('',#205424,#123321,#123322);
#103589=AXIS2_PLACEMENT_3D('',#205437,#123323,#123324);
#103590=AXIS2_PLACEMENT_3D('',#205450,#123325,#123326);
#103591=AXIS2_PLACEMENT_3D('',#205451,#123327,#123328);
#103592=AXIS2_PLACEMENT_3D('',#205452,#123329,#123330);
#103593=AXIS2_PLACEMENT_3D('',#205453,#123331,#123332);
#103594=AXIS2_PLACEMENT_3D('',#205454,#123333,#123334);
#103595=AXIS2_PLACEMENT_3D('',#205473,#123335,#123336);
#103596=AXIS2_PLACEMENT_3D('',#205474,#123337,#123338);
#103597=AXIS2_PLACEMENT_3D('',#205475,#123339,#123340);
#103598=AXIS2_PLACEMENT_3D('',#205476,#123341,#123342);
#103599=AXIS2_PLACEMENT_3D('',#205477,#123343,#123344);
#103600=AXIS2_PLACEMENT_3D('',#205490,#123345,#123346);
#103601=AXIS2_PLACEMENT_3D('',#205509,#123347,#123348);
#103602=AXIS2_PLACEMENT_3D('',#205510,#123349,#123350);
#103603=AXIS2_PLACEMENT_3D('',#205511,#123351,#123352);
#103604=AXIS2_PLACEMENT_3D('',#205512,#123353,#123354);
#103605=AXIS2_PLACEMENT_3D('',#205513,#123355,#123356);
#103606=AXIS2_PLACEMENT_3D('',#205532,#123357,#123358);
#103607=AXIS2_PLACEMENT_3D('',#205545,#123359,#123360);
#103608=AXIS2_PLACEMENT_3D('',#205546,#123361,#123362);
#103609=AXIS2_PLACEMENT_3D('',#205547,#123363,#123364);
#103610=AXIS2_PLACEMENT_3D('',#205548,#123365,#123366);
#103611=AXIS2_PLACEMENT_3D('',#205549,#123367,#123368);
#103612=AXIS2_PLACEMENT_3D('',#205568,#123369,#123370);
#103613=AXIS2_PLACEMENT_3D('',#205569,#123371,#123372);
#103614=AXIS2_PLACEMENT_3D('',#205570,#123373,#123374);
#103615=AXIS2_PLACEMENT_3D('',#205571,#123375,#123376);
#103616=AXIS2_PLACEMENT_3D('',#205572,#123377,#123378);
#103617=AXIS2_PLACEMENT_3D('',#205585,#123379,#123380);
#103618=AXIS2_PLACEMENT_3D('',#205598,#123381,#123382);
#103619=AXIS2_PLACEMENT_3D('',#205599,#123383,#123384);
#103620=AXIS2_PLACEMENT_3D('',#205600,#123385,#123386);
#103621=AXIS2_PLACEMENT_3D('',#205601,#123387,#123388);
#103622=AXIS2_PLACEMENT_3D('',#205602,#123389,#123390);
#103623=AXIS2_PLACEMENT_3D('',#205615,#123391,#123392);
#103624=AXIS2_PLACEMENT_3D('',#205616,#123393,#123394);
#103625=AXIS2_PLACEMENT_3D('',#205617,#123395,#123396);
#103626=AXIS2_PLACEMENT_3D('',#205618,#123397,#123398);
#103627=AXIS2_PLACEMENT_3D('',#205619,#123399,#123400);
#103628=AXIS2_PLACEMENT_3D('',#205632,#123401,#123402);
#103629=AXIS2_PLACEMENT_3D('',#205633,#123403,#123404);
#103630=AXIS2_PLACEMENT_3D('',#205634,#123405,#123406);
#103631=AXIS2_PLACEMENT_3D('',#205635,#123407,#123408);
#103632=AXIS2_PLACEMENT_3D('',#205636,#123409,#123410);
#103633=AXIS2_PLACEMENT_3D('',#205649,#123411,#123412);
#103634=AXIS2_PLACEMENT_3D('',#205662,#123413,#123414);
#103635=AXIS2_PLACEMENT_3D('',#205663,#123415,#123416);
#103636=AXIS2_PLACEMENT_3D('',#205664,#123417,#123418);
#103637=AXIS2_PLACEMENT_3D('',#205665,#123419,#123420);
#103638=AXIS2_PLACEMENT_3D('',#205666,#123421,#123422);
#103639=AXIS2_PLACEMENT_3D('',#205685,#123423,#123424);
#103640=AXIS2_PLACEMENT_3D('',#205686,#123425,#123426);
#103641=AXIS2_PLACEMENT_3D('',#205687,#123427,#123428);
#103642=AXIS2_PLACEMENT_3D('',#205688,#123429,#123430);
#103643=AXIS2_PLACEMENT_3D('',#205689,#123431,#123432);
#103644=AXIS2_PLACEMENT_3D('',#205702,#123433,#123434);
#103645=AXIS2_PLACEMENT_3D('',#205721,#123435,#123436);
#103646=AXIS2_PLACEMENT_3D('',#205722,#123437,#123438);
#103647=AXIS2_PLACEMENT_3D('',#205723,#123439,#123440);
#103648=AXIS2_PLACEMENT_3D('',#205724,#123441,#123442);
#103649=AXIS2_PLACEMENT_3D('',#205725,#123443,#123444);
#103650=AXIS2_PLACEMENT_3D('',#205744,#123445,#123446);
#103651=AXIS2_PLACEMENT_3D('',#205757,#123447,#123448);
#103652=AXIS2_PLACEMENT_3D('',#205758,#123449,#123450);
#103653=AXIS2_PLACEMENT_3D('',#205759,#123451,#123452);
#103654=AXIS2_PLACEMENT_3D('',#205760,#123453,#123454);
#103655=AXIS2_PLACEMENT_3D('',#205761,#123455,#123456);
#103656=AXIS2_PLACEMENT_3D('',#205780,#123457,#123458);
#103657=AXIS2_PLACEMENT_3D('',#205781,#123459,#123460);
#103658=AXIS2_PLACEMENT_3D('',#205782,#123461,#123462);
#103659=AXIS2_PLACEMENT_3D('',#205783,#123463,#123464);
#103660=AXIS2_PLACEMENT_3D('',#205784,#123465,#123466);
#103661=AXIS2_PLACEMENT_3D('',#205797,#123467,#123468);
#103662=AXIS2_PLACEMENT_3D('',#205810,#123469,#123470);
#103663=AXIS2_PLACEMENT_3D('',#205811,#123471,#123472);
#103664=AXIS2_PLACEMENT_3D('',#205812,#123473,#123474);
#103665=AXIS2_PLACEMENT_3D('',#205813,#123475,#123476);
#103666=AXIS2_PLACEMENT_3D('',#205814,#123477,#123478);
#103667=AXIS2_PLACEMENT_3D('',#205827,#123479,#123480);
#103668=AXIS2_PLACEMENT_3D('',#205828,#123481,#123482);
#103669=AXIS2_PLACEMENT_3D('',#205829,#123483,#123484);
#103670=AXIS2_PLACEMENT_3D('',#205830,#123485,#123486);
#103671=AXIS2_PLACEMENT_3D('',#205831,#123487,#123488);
#103672=AXIS2_PLACEMENT_3D('',#205844,#123489,#123490);
#103673=AXIS2_PLACEMENT_3D('',#205845,#123491,#123492);
#103674=AXIS2_PLACEMENT_3D('',#205846,#123493,#123494);
#103675=AXIS2_PLACEMENT_3D('',#205847,#123495,#123496);
#103676=AXIS2_PLACEMENT_3D('',#205848,#123497,#123498);
#103677=AXIS2_PLACEMENT_3D('',#205861,#123499,#123500);
#103678=AXIS2_PLACEMENT_3D('',#205874,#123501,#123502);
#103679=AXIS2_PLACEMENT_3D('',#205875,#123503,#123504);
#103680=AXIS2_PLACEMENT_3D('',#205876,#123505,#123506);
#103681=AXIS2_PLACEMENT_3D('',#205877,#123507,#123508);
#103682=AXIS2_PLACEMENT_3D('',#205878,#123509,#123510);
#103683=AXIS2_PLACEMENT_3D('',#205897,#123511,#123512);
#103684=AXIS2_PLACEMENT_3D('',#205898,#123513,#123514);
#103685=AXIS2_PLACEMENT_3D('',#205899,#123515,#123516);
#103686=AXIS2_PLACEMENT_3D('',#205900,#123517,#123518);
#103687=AXIS2_PLACEMENT_3D('',#205901,#123519,#123520);
#103688=AXIS2_PLACEMENT_3D('',#205914,#123521,#123522);
#103689=AXIS2_PLACEMENT_3D('',#205933,#123523,#123524);
#103690=AXIS2_PLACEMENT_3D('',#205934,#123525,#123526);
#103691=AXIS2_PLACEMENT_3D('',#205935,#123527,#123528);
#103692=AXIS2_PLACEMENT_3D('',#205936,#123529,#123530);
#103693=AXIS2_PLACEMENT_3D('',#205937,#123531,#123532);
#103694=AXIS2_PLACEMENT_3D('',#205956,#123533,#123534);
#103695=AXIS2_PLACEMENT_3D('',#205969,#123535,#123536);
#103696=AXIS2_PLACEMENT_3D('',#205970,#123537,#123538);
#103697=AXIS2_PLACEMENT_3D('',#205971,#123539,#123540);
#103698=AXIS2_PLACEMENT_3D('',#205972,#123541,#123542);
#103699=AXIS2_PLACEMENT_3D('',#205973,#123543,#123544);
#103700=AXIS2_PLACEMENT_3D('',#205992,#123545,#123546);
#103701=AXIS2_PLACEMENT_3D('',#205993,#123547,#123548);
#103702=AXIS2_PLACEMENT_3D('',#205994,#123549,#123550);
#103703=AXIS2_PLACEMENT_3D('',#205995,#123551,#123552);
#103704=AXIS2_PLACEMENT_3D('',#205996,#123553,#123554);
#103705=AXIS2_PLACEMENT_3D('',#206009,#123555,#123556);
#103706=AXIS2_PLACEMENT_3D('',#206022,#123557,#123558);
#103707=AXIS2_PLACEMENT_3D('',#206023,#123559,#123560);
#103708=AXIS2_PLACEMENT_3D('',#206024,#123561,#123562);
#103709=AXIS2_PLACEMENT_3D('',#206025,#123563,#123564);
#103710=AXIS2_PLACEMENT_3D('',#206026,#123565,#123566);
#103711=AXIS2_PLACEMENT_3D('',#206039,#123567,#123568);
#103712=AXIS2_PLACEMENT_3D('',#206040,#123569,#123570);
#103713=AXIS2_PLACEMENT_3D('',#206041,#123571,#123572);
#103714=AXIS2_PLACEMENT_3D('',#206042,#123573,#123574);
#103715=AXIS2_PLACEMENT_3D('',#206043,#123575,#123576);
#103716=AXIS2_PLACEMENT_3D('',#206056,#123577,#123578);
#103717=AXIS2_PLACEMENT_3D('',#206057,#123579,#123580);
#103718=AXIS2_PLACEMENT_3D('',#206058,#123581,#123582);
#103719=AXIS2_PLACEMENT_3D('',#206059,#123583,#123584);
#103720=AXIS2_PLACEMENT_3D('',#206060,#123585,#123586);
#103721=AXIS2_PLACEMENT_3D('',#206073,#123587,#123588);
#103722=AXIS2_PLACEMENT_3D('',#206086,#123589,#123590);
#103723=AXIS2_PLACEMENT_3D('',#206087,#123591,#123592);
#103724=AXIS2_PLACEMENT_3D('',#206088,#123593,#123594);
#103725=AXIS2_PLACEMENT_3D('',#206089,#123595,#123596);
#103726=AXIS2_PLACEMENT_3D('',#206090,#123597,#123598);
#103727=AXIS2_PLACEMENT_3D('',#206109,#123599,#123600);
#103728=AXIS2_PLACEMENT_3D('',#206110,#123601,#123602);
#103729=AXIS2_PLACEMENT_3D('',#206111,#123603,#123604);
#103730=AXIS2_PLACEMENT_3D('',#206112,#123605,#123606);
#103731=AXIS2_PLACEMENT_3D('',#206113,#123607,#123608);
#103732=AXIS2_PLACEMENT_3D('',#206126,#123609,#123610);
#103733=AXIS2_PLACEMENT_3D('',#206145,#123611,#123612);
#103734=AXIS2_PLACEMENT_3D('',#206146,#123613,#123614);
#103735=AXIS2_PLACEMENT_3D('',#206147,#123615,#123616);
#103736=AXIS2_PLACEMENT_3D('',#206148,#123617,#123618);
#103737=AXIS2_PLACEMENT_3D('',#206149,#123619,#123620);
#103738=AXIS2_PLACEMENT_3D('',#206168,#123621,#123622);
#103739=AXIS2_PLACEMENT_3D('',#206181,#123623,#123624);
#103740=AXIS2_PLACEMENT_3D('',#206182,#123625,#123626);
#103741=AXIS2_PLACEMENT_3D('',#206183,#123627,#123628);
#103742=AXIS2_PLACEMENT_3D('',#206184,#123629,#123630);
#103743=AXIS2_PLACEMENT_3D('',#206185,#123631,#123632);
#103744=AXIS2_PLACEMENT_3D('',#206204,#123633,#123634);
#103745=AXIS2_PLACEMENT_3D('',#206205,#123635,#123636);
#103746=AXIS2_PLACEMENT_3D('',#206206,#123637,#123638);
#103747=AXIS2_PLACEMENT_3D('',#206207,#123639,#123640);
#103748=AXIS2_PLACEMENT_3D('',#206208,#123641,#123642);
#103749=AXIS2_PLACEMENT_3D('',#206221,#123643,#123644);
#103750=AXIS2_PLACEMENT_3D('',#206234,#123645,#123646);
#103751=AXIS2_PLACEMENT_3D('',#206235,#123647,#123648);
#103752=AXIS2_PLACEMENT_3D('',#206236,#123649,#123650);
#103753=AXIS2_PLACEMENT_3D('',#206237,#123651,#123652);
#103754=AXIS2_PLACEMENT_3D('',#206238,#123653,#123654);
#103755=AXIS2_PLACEMENT_3D('',#206251,#123655,#123656);
#103756=AXIS2_PLACEMENT_3D('',#206252,#123657,#123658);
#103757=AXIS2_PLACEMENT_3D('',#206253,#123659,#123660);
#103758=AXIS2_PLACEMENT_3D('',#206254,#123661,#123662);
#103759=AXIS2_PLACEMENT_3D('',#206255,#123663,#123664);
#103760=AXIS2_PLACEMENT_3D('',#206268,#123665,#123666);
#103761=AXIS2_PLACEMENT_3D('',#206269,#123667,#123668);
#103762=AXIS2_PLACEMENT_3D('',#206270,#123669,#123670);
#103763=AXIS2_PLACEMENT_3D('',#206271,#123671,#123672);
#103764=AXIS2_PLACEMENT_3D('',#206272,#123673,#123674);
#103765=AXIS2_PLACEMENT_3D('',#206285,#123675,#123676);
#103766=AXIS2_PLACEMENT_3D('',#206298,#123677,#123678);
#103767=AXIS2_PLACEMENT_3D('',#206299,#123679,#123680);
#103768=AXIS2_PLACEMENT_3D('',#206300,#123681,#123682);
#103769=AXIS2_PLACEMENT_3D('',#206301,#123683,#123684);
#103770=AXIS2_PLACEMENT_3D('',#206302,#123685,#123686);
#103771=AXIS2_PLACEMENT_3D('',#206321,#123687,#123688);
#103772=AXIS2_PLACEMENT_3D('',#206322,#123689,#123690);
#103773=AXIS2_PLACEMENT_3D('',#206323,#123691,#123692);
#103774=AXIS2_PLACEMENT_3D('',#206324,#123693,#123694);
#103775=AXIS2_PLACEMENT_3D('',#206325,#123695,#123696);
#103776=AXIS2_PLACEMENT_3D('',#206338,#123697,#123698);
#103777=AXIS2_PLACEMENT_3D('',#206357,#123699,#123700);
#103778=AXIS2_PLACEMENT_3D('',#206358,#123701,#123702);
#103779=AXIS2_PLACEMENT_3D('',#206359,#123703,#123704);
#103780=AXIS2_PLACEMENT_3D('',#206360,#123705,#123706);
#103781=AXIS2_PLACEMENT_3D('',#206361,#123707,#123708);
#103782=AXIS2_PLACEMENT_3D('',#206380,#123709,#123710);
#103783=AXIS2_PLACEMENT_3D('',#206393,#123711,#123712);
#103784=AXIS2_PLACEMENT_3D('',#206394,#123713,#123714);
#103785=AXIS2_PLACEMENT_3D('',#206395,#123715,#123716);
#103786=AXIS2_PLACEMENT_3D('',#206396,#123717,#123718);
#103787=AXIS2_PLACEMENT_3D('',#206397,#123719,#123720);
#103788=AXIS2_PLACEMENT_3D('',#206416,#123721,#123722);
#103789=AXIS2_PLACEMENT_3D('',#206417,#123723,#123724);
#103790=AXIS2_PLACEMENT_3D('',#206418,#123725,#123726);
#103791=AXIS2_PLACEMENT_3D('',#206419,#123727,#123728);
#103792=AXIS2_PLACEMENT_3D('',#206420,#123729,#123730);
#103793=AXIS2_PLACEMENT_3D('',#206433,#123731,#123732);
#103794=AXIS2_PLACEMENT_3D('',#206446,#123733,#123734);
#103795=AXIS2_PLACEMENT_3D('',#206447,#123735,#123736);
#103796=AXIS2_PLACEMENT_3D('',#206448,#123737,#123738);
#103797=AXIS2_PLACEMENT_3D('',#206449,#123739,#123740);
#103798=AXIS2_PLACEMENT_3D('',#206450,#123741,#123742);
#103799=AXIS2_PLACEMENT_3D('',#206463,#123743,#123744);
#103800=AXIS2_PLACEMENT_3D('',#206464,#123745,#123746);
#103801=AXIS2_PLACEMENT_3D('',#206465,#123747,#123748);
#103802=AXIS2_PLACEMENT_3D('',#206466,#123749,#123750);
#103803=AXIS2_PLACEMENT_3D('',#206467,#123751,#123752);
#103804=AXIS2_PLACEMENT_3D('',#206480,#123753,#123754);
#103805=AXIS2_PLACEMENT_3D('',#206481,#123755,#123756);
#103806=AXIS2_PLACEMENT_3D('',#206482,#123757,#123758);
#103807=AXIS2_PLACEMENT_3D('',#206483,#123759,#123760);
#103808=AXIS2_PLACEMENT_3D('',#206484,#123761,#123762);
#103809=AXIS2_PLACEMENT_3D('',#206497,#123763,#123764);
#103810=AXIS2_PLACEMENT_3D('',#206510,#123765,#123766);
#103811=AXIS2_PLACEMENT_3D('',#206511,#123767,#123768);
#103812=AXIS2_PLACEMENT_3D('',#206512,#123769,#123770);
#103813=AXIS2_PLACEMENT_3D('',#206513,#123771,#123772);
#103814=AXIS2_PLACEMENT_3D('',#206514,#123773,#123774);
#103815=AXIS2_PLACEMENT_3D('',#206533,#123775,#123776);
#103816=AXIS2_PLACEMENT_3D('',#206534,#123777,#123778);
#103817=AXIS2_PLACEMENT_3D('',#206535,#123779,#123780);
#103818=AXIS2_PLACEMENT_3D('',#206536,#123781,#123782);
#103819=AXIS2_PLACEMENT_3D('',#206537,#123783,#123784);
#103820=AXIS2_PLACEMENT_3D('',#206550,#123785,#123786);
#103821=AXIS2_PLACEMENT_3D('',#206569,#123787,#123788);
#103822=AXIS2_PLACEMENT_3D('',#206570,#123789,#123790);
#103823=AXIS2_PLACEMENT_3D('',#206571,#123791,#123792);
#103824=AXIS2_PLACEMENT_3D('',#206572,#123793,#123794);
#103825=AXIS2_PLACEMENT_3D('',#206573,#123795,#123796);
#103826=AXIS2_PLACEMENT_3D('',#206592,#123797,#123798);
#103827=AXIS2_PLACEMENT_3D('',#206605,#123799,#123800);
#103828=AXIS2_PLACEMENT_3D('',#206606,#123801,#123802);
#103829=AXIS2_PLACEMENT_3D('',#206607,#123803,#123804);
#103830=AXIS2_PLACEMENT_3D('',#206608,#123805,#123806);
#103831=AXIS2_PLACEMENT_3D('',#206609,#123807,#123808);
#103832=AXIS2_PLACEMENT_3D('',#206628,#123809,#123810);
#103833=AXIS2_PLACEMENT_3D('',#206629,#123811,#123812);
#103834=AXIS2_PLACEMENT_3D('',#206630,#123813,#123814);
#103835=AXIS2_PLACEMENT_3D('',#206631,#123815,#123816);
#103836=AXIS2_PLACEMENT_3D('',#206632,#123817,#123818);
#103837=AXIS2_PLACEMENT_3D('',#206645,#123819,#123820);
#103838=AXIS2_PLACEMENT_3D('',#206658,#123821,#123822);
#103839=AXIS2_PLACEMENT_3D('',#206659,#123823,#123824);
#103840=AXIS2_PLACEMENT_3D('',#206660,#123825,#123826);
#103841=AXIS2_PLACEMENT_3D('',#206661,#123827,#123828);
#103842=AXIS2_PLACEMENT_3D('',#206662,#123829,#123830);
#103843=AXIS2_PLACEMENT_3D('',#206675,#123831,#123832);
#103844=AXIS2_PLACEMENT_3D('',#206676,#123833,#123834);
#103845=AXIS2_PLACEMENT_3D('',#206677,#123835,#123836);
#103846=AXIS2_PLACEMENT_3D('',#206678,#123837,#123838);
#103847=AXIS2_PLACEMENT_3D('',#206679,#123839,#123840);
#103848=AXIS2_PLACEMENT_3D('',#206692,#123841,#123842);
#103849=AXIS2_PLACEMENT_3D('',#206693,#123843,#123844);
#103850=AXIS2_PLACEMENT_3D('',#206694,#123845,#123846);
#103851=AXIS2_PLACEMENT_3D('',#206695,#123847,#123848);
#103852=AXIS2_PLACEMENT_3D('',#206696,#123849,#123850);
#103853=AXIS2_PLACEMENT_3D('',#206709,#123851,#123852);
#103854=AXIS2_PLACEMENT_3D('',#206722,#123853,#123854);
#103855=AXIS2_PLACEMENT_3D('',#206723,#123855,#123856);
#103856=AXIS2_PLACEMENT_3D('',#206724,#123857,#123858);
#103857=AXIS2_PLACEMENT_3D('',#206725,#123859,#123860);
#103858=AXIS2_PLACEMENT_3D('',#206726,#123861,#123862);
#103859=AXIS2_PLACEMENT_3D('',#206745,#123863,#123864);
#103860=AXIS2_PLACEMENT_3D('',#206746,#123865,#123866);
#103861=AXIS2_PLACEMENT_3D('',#206747,#123867,#123868);
#103862=AXIS2_PLACEMENT_3D('',#206748,#123869,#123870);
#103863=AXIS2_PLACEMENT_3D('',#206749,#123871,#123872);
#103864=AXIS2_PLACEMENT_3D('',#206762,#123873,#123874);
#103865=AXIS2_PLACEMENT_3D('',#206781,#123875,#123876);
#103866=AXIS2_PLACEMENT_3D('',#206782,#123877,#123878);
#103867=AXIS2_PLACEMENT_3D('',#206783,#123879,#123880);
#103868=AXIS2_PLACEMENT_3D('',#206784,#123881,#123882);
#103869=AXIS2_PLACEMENT_3D('',#206785,#123883,#123884);
#103870=AXIS2_PLACEMENT_3D('',#206804,#123885,#123886);
#103871=AXIS2_PLACEMENT_3D('',#206817,#123887,#123888);
#103872=AXIS2_PLACEMENT_3D('',#206818,#123889,#123890);
#103873=AXIS2_PLACEMENT_3D('',#206819,#123891,#123892);
#103874=AXIS2_PLACEMENT_3D('',#206820,#123893,#123894);
#103875=AXIS2_PLACEMENT_3D('',#206821,#123895,#123896);
#103876=AXIS2_PLACEMENT_3D('',#206840,#123897,#123898);
#103877=AXIS2_PLACEMENT_3D('',#206841,#123899,#123900);
#103878=AXIS2_PLACEMENT_3D('',#206842,#123901,#123902);
#103879=AXIS2_PLACEMENT_3D('',#206843,#123903,#123904);
#103880=AXIS2_PLACEMENT_3D('',#206844,#123905,#123906);
#103881=AXIS2_PLACEMENT_3D('',#206857,#123907,#123908);
#103882=AXIS2_PLACEMENT_3D('',#206870,#123909,#123910);
#103883=AXIS2_PLACEMENT_3D('',#206871,#123911,#123912);
#103884=AXIS2_PLACEMENT_3D('',#206872,#123913,#123914);
#103885=AXIS2_PLACEMENT_3D('',#206873,#123915,#123916);
#103886=AXIS2_PLACEMENT_3D('',#206874,#123917,#123918);
#103887=AXIS2_PLACEMENT_3D('',#206887,#123919,#123920);
#103888=AXIS2_PLACEMENT_3D('',#206888,#123921,#123922);
#103889=AXIS2_PLACEMENT_3D('',#206889,#123923,#123924);
#103890=AXIS2_PLACEMENT_3D('',#206890,#123925,#123926);
#103891=AXIS2_PLACEMENT_3D('',#206891,#123927,#123928);
#103892=AXIS2_PLACEMENT_3D('',#206904,#123929,#123930);
#103893=AXIS2_PLACEMENT_3D('',#206905,#123931,#123932);
#103894=AXIS2_PLACEMENT_3D('',#206906,#123933,#123934);
#103895=AXIS2_PLACEMENT_3D('',#206907,#123935,#123936);
#103896=AXIS2_PLACEMENT_3D('',#206908,#123937,#123938);
#103897=AXIS2_PLACEMENT_3D('',#206921,#123939,#123940);
#103898=AXIS2_PLACEMENT_3D('',#206934,#123941,#123942);
#103899=AXIS2_PLACEMENT_3D('',#206935,#123943,#123944);
#103900=AXIS2_PLACEMENT_3D('',#206936,#123945,#123946);
#103901=AXIS2_PLACEMENT_3D('',#206937,#123947,#123948);
#103902=AXIS2_PLACEMENT_3D('',#206938,#123949,#123950);
#103903=AXIS2_PLACEMENT_3D('',#206957,#123951,#123952);
#103904=AXIS2_PLACEMENT_3D('',#206958,#123953,#123954);
#103905=AXIS2_PLACEMENT_3D('',#206959,#123955,#123956);
#103906=AXIS2_PLACEMENT_3D('',#206960,#123957,#123958);
#103907=AXIS2_PLACEMENT_3D('',#206961,#123959,#123960);
#103908=AXIS2_PLACEMENT_3D('',#206974,#123961,#123962);
#103909=AXIS2_PLACEMENT_3D('',#206993,#123963,#123964);
#103910=AXIS2_PLACEMENT_3D('',#206994,#123965,#123966);
#103911=AXIS2_PLACEMENT_3D('',#206995,#123967,#123968);
#103912=AXIS2_PLACEMENT_3D('',#206996,#123969,#123970);
#103913=AXIS2_PLACEMENT_3D('',#206997,#123971,#123972);
#103914=AXIS2_PLACEMENT_3D('',#207016,#123973,#123974);
#103915=AXIS2_PLACEMENT_3D('',#207029,#123975,#123976);
#103916=AXIS2_PLACEMENT_3D('',#207030,#123977,#123978);
#103917=AXIS2_PLACEMENT_3D('',#207031,#123979,#123980);
#103918=AXIS2_PLACEMENT_3D('',#207032,#123981,#123982);
#103919=AXIS2_PLACEMENT_3D('',#207033,#123983,#123984);
#103920=AXIS2_PLACEMENT_3D('',#207052,#123985,#123986);
#103921=AXIS2_PLACEMENT_3D('',#207053,#123987,#123988);
#103922=AXIS2_PLACEMENT_3D('',#207054,#123989,#123990);
#103923=AXIS2_PLACEMENT_3D('',#207055,#123991,#123992);
#103924=AXIS2_PLACEMENT_3D('',#207056,#123993,#123994);
#103925=AXIS2_PLACEMENT_3D('',#207069,#123995,#123996);
#103926=AXIS2_PLACEMENT_3D('',#207082,#123997,#123998);
#103927=AXIS2_PLACEMENT_3D('',#207083,#123999,#124000);
#103928=AXIS2_PLACEMENT_3D('',#207084,#124001,#124002);
#103929=AXIS2_PLACEMENT_3D('',#207085,#124003,#124004);
#103930=AXIS2_PLACEMENT_3D('',#207086,#124005,#124006);
#103931=AXIS2_PLACEMENT_3D('',#207099,#124007,#124008);
#103932=AXIS2_PLACEMENT_3D('',#207100,#124009,#124010);
#103933=AXIS2_PLACEMENT_3D('',#207101,#124011,#124012);
#103934=AXIS2_PLACEMENT_3D('',#207102,#124013,#124014);
#103935=AXIS2_PLACEMENT_3D('',#207103,#124015,#124016);
#103936=AXIS2_PLACEMENT_3D('',#207116,#124017,#124018);
#103937=AXIS2_PLACEMENT_3D('',#207117,#124019,#124020);
#103938=AXIS2_PLACEMENT_3D('',#207118,#124021,#124022);
#103939=AXIS2_PLACEMENT_3D('',#207119,#124023,#124024);
#103940=AXIS2_PLACEMENT_3D('',#207120,#124025,#124026);
#103941=AXIS2_PLACEMENT_3D('',#207133,#124027,#124028);
#103942=AXIS2_PLACEMENT_3D('',#207146,#124029,#124030);
#103943=AXIS2_PLACEMENT_3D('',#207147,#124031,#124032);
#103944=AXIS2_PLACEMENT_3D('',#207148,#124033,#124034);
#103945=AXIS2_PLACEMENT_3D('',#207149,#124035,#124036);
#103946=AXIS2_PLACEMENT_3D('',#207150,#124037,#124038);
#103947=AXIS2_PLACEMENT_3D('',#207169,#124039,#124040);
#103948=AXIS2_PLACEMENT_3D('',#207170,#124041,#124042);
#103949=AXIS2_PLACEMENT_3D('',#207171,#124043,#124044);
#103950=AXIS2_PLACEMENT_3D('',#207172,#124045,#124046);
#103951=AXIS2_PLACEMENT_3D('',#207173,#124047,#124048);
#103952=AXIS2_PLACEMENT_3D('',#207186,#124049,#124050);
#103953=AXIS2_PLACEMENT_3D('',#207205,#124051,#124052);
#103954=AXIS2_PLACEMENT_3D('',#207206,#124053,#124054);
#103955=AXIS2_PLACEMENT_3D('',#207207,#124055,#124056);
#103956=AXIS2_PLACEMENT_3D('',#207208,#124057,#124058);
#103957=AXIS2_PLACEMENT_3D('',#207209,#124059,#124060);
#103958=AXIS2_PLACEMENT_3D('',#207228,#124061,#124062);
#103959=AXIS2_PLACEMENT_3D('',#207241,#124063,#124064);
#103960=AXIS2_PLACEMENT_3D('',#207242,#124065,#124066);
#103961=AXIS2_PLACEMENT_3D('',#207243,#124067,#124068);
#103962=AXIS2_PLACEMENT_3D('',#207244,#124069,#124070);
#103963=AXIS2_PLACEMENT_3D('',#207245,#124071,#124072);
#103964=AXIS2_PLACEMENT_3D('',#207264,#124073,#124074);
#103965=AXIS2_PLACEMENT_3D('',#207265,#124075,#124076);
#103966=AXIS2_PLACEMENT_3D('',#207266,#124077,#124078);
#103967=AXIS2_PLACEMENT_3D('',#207267,#124079,#124080);
#103968=AXIS2_PLACEMENT_3D('',#207268,#124081,#124082);
#103969=AXIS2_PLACEMENT_3D('',#207281,#124083,#124084);
#103970=AXIS2_PLACEMENT_3D('',#207294,#124085,#124086);
#103971=AXIS2_PLACEMENT_3D('',#207295,#124087,#124088);
#103972=AXIS2_PLACEMENT_3D('',#207296,#124089,#124090);
#103973=AXIS2_PLACEMENT_3D('',#207297,#124091,#124092);
#103974=AXIS2_PLACEMENT_3D('',#207298,#124093,#124094);
#103975=AXIS2_PLACEMENT_3D('',#207311,#124095,#124096);
#103976=AXIS2_PLACEMENT_3D('',#207312,#124097,#124098);
#103977=AXIS2_PLACEMENT_3D('',#207313,#124099,#124100);
#103978=AXIS2_PLACEMENT_3D('',#207314,#124101,#124102);
#103979=AXIS2_PLACEMENT_3D('',#207315,#124103,#124104);
#103980=AXIS2_PLACEMENT_3D('',#207328,#124105,#124106);
#103981=AXIS2_PLACEMENT_3D('',#207329,#124107,#124108);
#103982=AXIS2_PLACEMENT_3D('',#207330,#124109,#124110);
#103983=AXIS2_PLACEMENT_3D('',#207331,#124111,#124112);
#103984=AXIS2_PLACEMENT_3D('',#207332,#124113,#124114);
#103985=AXIS2_PLACEMENT_3D('',#207345,#124115,#124116);
#103986=AXIS2_PLACEMENT_3D('',#207358,#124117,#124118);
#103987=AXIS2_PLACEMENT_3D('',#207359,#124119,#124120);
#103988=AXIS2_PLACEMENT_3D('',#207360,#124121,#124122);
#103989=AXIS2_PLACEMENT_3D('',#207361,#124123,#124124);
#103990=AXIS2_PLACEMENT_3D('',#207362,#124125,#124126);
#103991=AXIS2_PLACEMENT_3D('',#207381,#124127,#124128);
#103992=AXIS2_PLACEMENT_3D('',#207382,#124129,#124130);
#103993=AXIS2_PLACEMENT_3D('',#207395,#124131,#124132);
#103994=AXIS2_PLACEMENT_3D('',#207414,#124133,#124134);
#103995=AXIS2_PLACEMENT_3D('',#207415,#124135,#124136);
#103996=AXIS2_PLACEMENT_3D('',#207416,#124137,#124138);
#103997=AXIS2_PLACEMENT_3D('',#207417,#124139,#124140);
#103998=AXIS2_PLACEMENT_3D('',#207418,#124141,#124142);
#103999=AXIS2_PLACEMENT_3D('',#207449,#124143,#124144);
#104000=AXIS2_PLACEMENT_3D('',#207450,#124145,#124146);
#104001=AXIS2_PLACEMENT_3D('',#207451,#124147,#124148);
#104002=AXIS2_PLACEMENT_3D('',#207470,#124149,#124150);
#104003=AXIS2_PLACEMENT_3D('',#207471,#124151,#124152);
#104004=AXIS2_PLACEMENT_3D('',#207472,#124153,#124154);
#104005=AXIS2_PLACEMENT_3D('',#207473,#124155,#124156);
#104006=AXIS2_PLACEMENT_3D('',#207474,#124157,#124158);
#104007=AXIS2_PLACEMENT_3D('',#207487,#124159,#124160);
#104008=AXIS2_PLACEMENT_3D('',#207500,#124161,#124162);
#104009=AXIS2_PLACEMENT_3D('',#207501,#124163,#124164);
#104010=AXIS2_PLACEMENT_3D('',#207502,#124165,#124166);
#104011=AXIS2_PLACEMENT_3D('',#207503,#124167,#124168);
#104012=AXIS2_PLACEMENT_3D('',#207504,#124169,#124170);
#104013=AXIS2_PLACEMENT_3D('',#207517,#124171,#124172);
#104014=AXIS2_PLACEMENT_3D('',#207518,#124173,#124174);
#104015=AXIS2_PLACEMENT_3D('',#207519,#124175,#124176);
#104016=AXIS2_PLACEMENT_3D('',#207520,#124177,#124178);
#104017=AXIS2_PLACEMENT_3D('',#207521,#124179,#124180);
#104018=AXIS2_PLACEMENT_3D('',#207534,#124181,#124182);
#104019=AXIS2_PLACEMENT_3D('',#207535,#124183,#124184);
#104020=AXIS2_PLACEMENT_3D('',#207536,#124185,#124186);
#104021=AXIS2_PLACEMENT_3D('',#207537,#124187,#124188);
#104022=AXIS2_PLACEMENT_3D('',#207538,#124189,#124190);
#104023=AXIS2_PLACEMENT_3D('',#207551,#124191,#124192);
#104024=AXIS2_PLACEMENT_3D('',#207564,#124193,#124194);
#104025=AXIS2_PLACEMENT_3D('',#207565,#124195,#124196);
#104026=AXIS2_PLACEMENT_3D('',#207566,#124197,#124198);
#104027=AXIS2_PLACEMENT_3D('',#207567,#124199,#124200);
#104028=AXIS2_PLACEMENT_3D('',#207568,#124201,#124202);
#104029=AXIS2_PLACEMENT_3D('',#207587,#124203,#124204);
#104030=AXIS2_PLACEMENT_3D('',#207588,#124205,#124206);
#104031=AXIS2_PLACEMENT_3D('',#207589,#124207,#124208);
#104032=AXIS2_PLACEMENT_3D('',#207590,#124209,#124210);
#104033=AXIS2_PLACEMENT_3D('',#207591,#124211,#124212);
#104034=AXIS2_PLACEMENT_3D('',#207604,#124213,#124214);
#104035=AXIS2_PLACEMENT_3D('',#207623,#124215,#124216);
#104036=AXIS2_PLACEMENT_3D('',#207624,#124217,#124218);
#104037=AXIS2_PLACEMENT_3D('',#207625,#124219,#124220);
#104038=AXIS2_PLACEMENT_3D('',#207626,#124221,#124222);
#104039=AXIS2_PLACEMENT_3D('',#207627,#124223,#124224);
#104040=AXIS2_PLACEMENT_3D('',#207646,#124225,#124226);
#104041=AXIS2_PLACEMENT_3D('',#207659,#124227,#124228);
#104042=AXIS2_PLACEMENT_3D('',#207660,#124229,#124230);
#104043=AXIS2_PLACEMENT_3D('',#207661,#124231,#124232);
#104044=AXIS2_PLACEMENT_3D('',#207662,#124233,#124234);
#104045=AXIS2_PLACEMENT_3D('',#207663,#124235,#124236);
#104046=AXIS2_PLACEMENT_3D('',#207682,#124237,#124238);
#104047=AXIS2_PLACEMENT_3D('',#207683,#124239,#124240);
#104048=AXIS2_PLACEMENT_3D('',#207684,#124241,#124242);
#104049=AXIS2_PLACEMENT_3D('',#207685,#124243,#124244);
#104050=AXIS2_PLACEMENT_3D('',#207686,#124245,#124246);
#104051=AXIS2_PLACEMENT_3D('',#207699,#124247,#124248);
#104052=AXIS2_PLACEMENT_3D('',#207712,#124249,#124250);
#104053=AXIS2_PLACEMENT_3D('',#207713,#124251,#124252);
#104054=AXIS2_PLACEMENT_3D('',#207714,#124253,#124254);
#104055=AXIS2_PLACEMENT_3D('',#207715,#124255,#124256);
#104056=AXIS2_PLACEMENT_3D('',#207716,#124257,#124258);
#104057=AXIS2_PLACEMENT_3D('',#207729,#124259,#124260);
#104058=AXIS2_PLACEMENT_3D('',#207730,#124261,#124262);
#104059=AXIS2_PLACEMENT_3D('',#207731,#124263,#124264);
#104060=AXIS2_PLACEMENT_3D('',#207732,#124265,#124266);
#104061=AXIS2_PLACEMENT_3D('',#207733,#124267,#124268);
#104062=AXIS2_PLACEMENT_3D('',#207746,#124269,#124270);
#104063=AXIS2_PLACEMENT_3D('',#207747,#124271,#124272);
#104064=AXIS2_PLACEMENT_3D('',#207748,#124273,#124274);
#104065=AXIS2_PLACEMENT_3D('',#207749,#124275,#124276);
#104066=AXIS2_PLACEMENT_3D('',#207750,#124277,#124278);
#104067=AXIS2_PLACEMENT_3D('',#207763,#124279,#124280);
#104068=AXIS2_PLACEMENT_3D('',#207776,#124281,#124282);
#104069=AXIS2_PLACEMENT_3D('',#207777,#124283,#124284);
#104070=AXIS2_PLACEMENT_3D('',#207778,#124285,#124286);
#104071=AXIS2_PLACEMENT_3D('',#207779,#124287,#124288);
#104072=AXIS2_PLACEMENT_3D('',#207780,#124289,#124290);
#104073=AXIS2_PLACEMENT_3D('',#207799,#124291,#124292);
#104074=AXIS2_PLACEMENT_3D('',#207800,#124293,#124294);
#104075=AXIS2_PLACEMENT_3D('',#207801,#124295,#124296);
#104076=AXIS2_PLACEMENT_3D('',#207802,#124297,#124298);
#104077=AXIS2_PLACEMENT_3D('',#207803,#124299,#124300);
#104078=AXIS2_PLACEMENT_3D('',#207816,#124301,#124302);
#104079=AXIS2_PLACEMENT_3D('',#207835,#124303,#124304);
#104080=AXIS2_PLACEMENT_3D('',#207836,#124305,#124306);
#104081=AXIS2_PLACEMENT_3D('',#207837,#124307,#124308);
#104082=AXIS2_PLACEMENT_3D('',#207838,#124309,#124310);
#104083=AXIS2_PLACEMENT_3D('',#207839,#124311,#124312);
#104084=AXIS2_PLACEMENT_3D('',#207858,#124313,#124314);
#104085=AXIS2_PLACEMENT_3D('',#207871,#124315,#124316);
#104086=AXIS2_PLACEMENT_3D('',#207872,#124317,#124318);
#104087=AXIS2_PLACEMENT_3D('',#207873,#124319,#124320);
#104088=AXIS2_PLACEMENT_3D('',#207874,#124321,#124322);
#104089=AXIS2_PLACEMENT_3D('',#207875,#124323,#124324);
#104090=AXIS2_PLACEMENT_3D('',#207894,#124325,#124326);
#104091=AXIS2_PLACEMENT_3D('',#207895,#124327,#124328);
#104092=AXIS2_PLACEMENT_3D('',#207896,#124329,#124330);
#104093=AXIS2_PLACEMENT_3D('',#207897,#124331,#124332);
#104094=AXIS2_PLACEMENT_3D('',#207898,#124333,#124334);
#104095=AXIS2_PLACEMENT_3D('',#207911,#124335,#124336);
#104096=AXIS2_PLACEMENT_3D('',#207924,#124337,#124338);
#104097=AXIS2_PLACEMENT_3D('',#207925,#124339,#124340);
#104098=AXIS2_PLACEMENT_3D('',#207926,#124341,#124342);
#104099=AXIS2_PLACEMENT_3D('',#207927,#124343,#124344);
#104100=AXIS2_PLACEMENT_3D('',#207928,#124345,#124346);
#104101=AXIS2_PLACEMENT_3D('',#207941,#124347,#124348);
#104102=AXIS2_PLACEMENT_3D('',#207942,#124349,#124350);
#104103=AXIS2_PLACEMENT_3D('',#207943,#124351,#124352);
#104104=AXIS2_PLACEMENT_3D('',#207944,#124353,#124354);
#104105=AXIS2_PLACEMENT_3D('',#207945,#124355,#124356);
#104106=AXIS2_PLACEMENT_3D('',#207958,#124357,#124358);
#104107=AXIS2_PLACEMENT_3D('',#207959,#124359,#124360);
#104108=AXIS2_PLACEMENT_3D('',#207960,#124361,#124362);
#104109=AXIS2_PLACEMENT_3D('',#207961,#124363,#124364);
#104110=AXIS2_PLACEMENT_3D('',#207962,#124365,#124366);
#104111=AXIS2_PLACEMENT_3D('',#207975,#124367,#124368);
#104112=AXIS2_PLACEMENT_3D('',#207988,#124369,#124370);
#104113=AXIS2_PLACEMENT_3D('',#207989,#124371,#124372);
#104114=AXIS2_PLACEMENT_3D('',#207990,#124373,#124374);
#104115=AXIS2_PLACEMENT_3D('',#207991,#124375,#124376);
#104116=AXIS2_PLACEMENT_3D('',#207992,#124377,#124378);
#104117=AXIS2_PLACEMENT_3D('',#208011,#124379,#124380);
#104118=AXIS2_PLACEMENT_3D('',#208012,#124381,#124382);
#104119=AXIS2_PLACEMENT_3D('',#208013,#124383,#124384);
#104120=AXIS2_PLACEMENT_3D('',#208014,#124385,#124386);
#104121=AXIS2_PLACEMENT_3D('',#208015,#124387,#124388);
#104122=AXIS2_PLACEMENT_3D('',#208028,#124389,#124390);
#104123=AXIS2_PLACEMENT_3D('',#208047,#124391,#124392);
#104124=AXIS2_PLACEMENT_3D('',#208048,#124393,#124394);
#104125=AXIS2_PLACEMENT_3D('',#208049,#124395,#124396);
#104126=AXIS2_PLACEMENT_3D('',#208050,#124397,#124398);
#104127=AXIS2_PLACEMENT_3D('',#208051,#124399,#124400);
#104128=AXIS2_PLACEMENT_3D('',#208070,#124401,#124402);
#104129=AXIS2_PLACEMENT_3D('',#208083,#124403,#124404);
#104130=AXIS2_PLACEMENT_3D('',#208084,#124405,#124406);
#104131=AXIS2_PLACEMENT_3D('',#208085,#124407,#124408);
#104132=AXIS2_PLACEMENT_3D('',#208086,#124409,#124410);
#104133=AXIS2_PLACEMENT_3D('',#208087,#124411,#124412);
#104134=AXIS2_PLACEMENT_3D('',#208106,#124413,#124414);
#104135=AXIS2_PLACEMENT_3D('',#208107,#124415,#124416);
#104136=AXIS2_PLACEMENT_3D('',#208108,#124417,#124418);
#104137=AXIS2_PLACEMENT_3D('',#208109,#124419,#124420);
#104138=AXIS2_PLACEMENT_3D('',#208110,#124421,#124422);
#104139=AXIS2_PLACEMENT_3D('',#208123,#124423,#124424);
#104140=AXIS2_PLACEMENT_3D('',#208136,#124425,#124426);
#104141=AXIS2_PLACEMENT_3D('',#208137,#124427,#124428);
#104142=AXIS2_PLACEMENT_3D('',#208138,#124429,#124430);
#104143=AXIS2_PLACEMENT_3D('',#208139,#124431,#124432);
#104144=AXIS2_PLACEMENT_3D('',#208140,#124433,#124434);
#104145=AXIS2_PLACEMENT_3D('',#208153,#124435,#124436);
#104146=AXIS2_PLACEMENT_3D('',#208154,#124437,#124438);
#104147=AXIS2_PLACEMENT_3D('',#208155,#124439,#124440);
#104148=AXIS2_PLACEMENT_3D('',#208156,#124441,#124442);
#104149=AXIS2_PLACEMENT_3D('',#208157,#124443,#124444);
#104150=AXIS2_PLACEMENT_3D('',#208170,#124445,#124446);
#104151=AXIS2_PLACEMENT_3D('',#208171,#124447,#124448);
#104152=AXIS2_PLACEMENT_3D('',#208172,#124449,#124450);
#104153=AXIS2_PLACEMENT_3D('',#208173,#124451,#124452);
#104154=AXIS2_PLACEMENT_3D('',#208174,#124453,#124454);
#104155=AXIS2_PLACEMENT_3D('',#208187,#124455,#124456);
#104156=AXIS2_PLACEMENT_3D('',#208200,#124457,#124458);
#104157=AXIS2_PLACEMENT_3D('',#208201,#124459,#124460);
#104158=AXIS2_PLACEMENT_3D('',#208202,#124461,#124462);
#104159=AXIS2_PLACEMENT_3D('',#208203,#124463,#124464);
#104160=AXIS2_PLACEMENT_3D('',#208204,#124465,#124466);
#104161=AXIS2_PLACEMENT_3D('',#208223,#124467,#124468);
#104162=AXIS2_PLACEMENT_3D('',#208224,#124469,#124470);
#104163=AXIS2_PLACEMENT_3D('',#208225,#124471,#124472);
#104164=AXIS2_PLACEMENT_3D('',#208226,#124473,#124474);
#104165=AXIS2_PLACEMENT_3D('',#208227,#124475,#124476);
#104166=AXIS2_PLACEMENT_3D('',#208240,#124477,#124478);
#104167=AXIS2_PLACEMENT_3D('',#208259,#124479,#124480);
#104168=AXIS2_PLACEMENT_3D('',#208260,#124481,#124482);
#104169=AXIS2_PLACEMENT_3D('',#208261,#124483,#124484);
#104170=AXIS2_PLACEMENT_3D('',#208262,#124485,#124486);
#104171=AXIS2_PLACEMENT_3D('',#208263,#124487,#124488);
#104172=AXIS2_PLACEMENT_3D('',#208282,#124489,#124490);
#104173=AXIS2_PLACEMENT_3D('',#208295,#124491,#124492);
#104174=AXIS2_PLACEMENT_3D('',#208296,#124493,#124494);
#104175=AXIS2_PLACEMENT_3D('',#208297,#124495,#124496);
#104176=AXIS2_PLACEMENT_3D('',#208298,#124497,#124498);
#104177=AXIS2_PLACEMENT_3D('',#208299,#124499,#124500);
#104178=AXIS2_PLACEMENT_3D('',#208318,#124501,#124502);
#104179=AXIS2_PLACEMENT_3D('',#208319,#124503,#124504);
#104180=AXIS2_PLACEMENT_3D('',#208320,#124505,#124506);
#104181=AXIS2_PLACEMENT_3D('',#208321,#124507,#124508);
#104182=AXIS2_PLACEMENT_3D('',#208322,#124509,#124510);
#104183=AXIS2_PLACEMENT_3D('',#208335,#124511,#124512);
#104184=AXIS2_PLACEMENT_3D('',#208348,#124513,#124514);
#104185=AXIS2_PLACEMENT_3D('',#208349,#124515,#124516);
#104186=AXIS2_PLACEMENT_3D('',#208350,#124517,#124518);
#104187=AXIS2_PLACEMENT_3D('',#208351,#124519,#124520);
#104188=AXIS2_PLACEMENT_3D('',#208352,#124521,#124522);
#104189=AXIS2_PLACEMENT_3D('',#208365,#124523,#124524);
#104190=AXIS2_PLACEMENT_3D('',#208366,#124525,#124526);
#104191=AXIS2_PLACEMENT_3D('',#208367,#124527,#124528);
#104192=AXIS2_PLACEMENT_3D('',#208368,#124529,#124530);
#104193=AXIS2_PLACEMENT_3D('',#208369,#124531,#124532);
#104194=AXIS2_PLACEMENT_3D('',#208382,#124533,#124534);
#104195=AXIS2_PLACEMENT_3D('',#208383,#124535,#124536);
#104196=AXIS2_PLACEMENT_3D('',#208384,#124537,#124538);
#104197=AXIS2_PLACEMENT_3D('',#208385,#124539,#124540);
#104198=AXIS2_PLACEMENT_3D('',#208386,#124541,#124542);
#104199=AXIS2_PLACEMENT_3D('',#208399,#124543,#124544);
#104200=AXIS2_PLACEMENT_3D('',#208412,#124545,#124546);
#104201=AXIS2_PLACEMENT_3D('',#208413,#124547,#124548);
#104202=AXIS2_PLACEMENT_3D('',#208414,#124549,#124550);
#104203=AXIS2_PLACEMENT_3D('',#208415,#124551,#124552);
#104204=AXIS2_PLACEMENT_3D('',#208416,#124553,#124554);
#104205=AXIS2_PLACEMENT_3D('',#208435,#124555,#124556);
#104206=AXIS2_PLACEMENT_3D('',#208436,#124557,#124558);
#104207=AXIS2_PLACEMENT_3D('',#208437,#124559,#124560);
#104208=AXIS2_PLACEMENT_3D('',#208438,#124561,#124562);
#104209=AXIS2_PLACEMENT_3D('',#208439,#124563,#124564);
#104210=AXIS2_PLACEMENT_3D('',#208452,#124565,#124566);
#104211=AXIS2_PLACEMENT_3D('',#208471,#124567,#124568);
#104212=AXIS2_PLACEMENT_3D('',#208472,#124569,#124570);
#104213=AXIS2_PLACEMENT_3D('',#208473,#124571,#124572);
#104214=AXIS2_PLACEMENT_3D('',#208474,#124573,#124574);
#104215=AXIS2_PLACEMENT_3D('',#208475,#124575,#124576);
#104216=AXIS2_PLACEMENT_3D('',#208494,#124577,#124578);
#104217=AXIS2_PLACEMENT_3D('',#208507,#124579,#124580);
#104218=AXIS2_PLACEMENT_3D('',#208508,#124581,#124582);
#104219=AXIS2_PLACEMENT_3D('',#208509,#124583,#124584);
#104220=AXIS2_PLACEMENT_3D('',#208510,#124585,#124586);
#104221=AXIS2_PLACEMENT_3D('',#208511,#124587,#124588);
#104222=AXIS2_PLACEMENT_3D('',#208530,#124589,#124590);
#104223=AXIS2_PLACEMENT_3D('',#208531,#124591,#124592);
#104224=AXIS2_PLACEMENT_3D('',#208532,#124593,#124594);
#104225=AXIS2_PLACEMENT_3D('',#208533,#124595,#124596);
#104226=AXIS2_PLACEMENT_3D('',#208534,#124597,#124598);
#104227=AXIS2_PLACEMENT_3D('',#208547,#124599,#124600);
#104228=AXIS2_PLACEMENT_3D('',#208560,#124601,#124602);
#104229=AXIS2_PLACEMENT_3D('',#208561,#124603,#124604);
#104230=AXIS2_PLACEMENT_3D('',#208562,#124605,#124606);
#104231=AXIS2_PLACEMENT_3D('',#208563,#124607,#124608);
#104232=AXIS2_PLACEMENT_3D('',#208564,#124609,#124610);
#104233=AXIS2_PLACEMENT_3D('',#208577,#124611,#124612);
#104234=AXIS2_PLACEMENT_3D('',#208578,#124613,#124614);
#104235=AXIS2_PLACEMENT_3D('',#208579,#124615,#124616);
#104236=AXIS2_PLACEMENT_3D('',#208580,#124617,#124618);
#104237=AXIS2_PLACEMENT_3D('',#208581,#124619,#124620);
#104238=AXIS2_PLACEMENT_3D('',#208594,#124621,#124622);
#104239=AXIS2_PLACEMENT_3D('',#208595,#124623,#124624);
#104240=AXIS2_PLACEMENT_3D('',#208596,#124625,#124626);
#104241=AXIS2_PLACEMENT_3D('',#208597,#124627,#124628);
#104242=AXIS2_PLACEMENT_3D('',#208598,#124629,#124630);
#104243=AXIS2_PLACEMENT_3D('',#208611,#124631,#124632);
#104244=AXIS2_PLACEMENT_3D('',#208624,#124633,#124634);
#104245=AXIS2_PLACEMENT_3D('',#208625,#124635,#124636);
#104246=AXIS2_PLACEMENT_3D('',#208626,#124637,#124638);
#104247=AXIS2_PLACEMENT_3D('',#208627,#124639,#124640);
#104248=AXIS2_PLACEMENT_3D('',#208628,#124641,#124642);
#104249=AXIS2_PLACEMENT_3D('',#208647,#124643,#124644);
#104250=AXIS2_PLACEMENT_3D('',#208648,#124645,#124646);
#104251=AXIS2_PLACEMENT_3D('',#208649,#124647,#124648);
#104252=AXIS2_PLACEMENT_3D('',#208650,#124649,#124650);
#104253=AXIS2_PLACEMENT_3D('',#208651,#124651,#124652);
#104254=AXIS2_PLACEMENT_3D('',#208664,#124653,#124654);
#104255=AXIS2_PLACEMENT_3D('',#208683,#124655,#124656);
#104256=AXIS2_PLACEMENT_3D('',#208684,#124657,#124658);
#104257=AXIS2_PLACEMENT_3D('',#208685,#124659,#124660);
#104258=AXIS2_PLACEMENT_3D('',#208686,#124661,#124662);
#104259=AXIS2_PLACEMENT_3D('',#208687,#124663,#124664);
#104260=AXIS2_PLACEMENT_3D('',#208706,#124665,#124666);
#104261=AXIS2_PLACEMENT_3D('',#208719,#124667,#124668);
#104262=AXIS2_PLACEMENT_3D('',#208720,#124669,#124670);
#104263=AXIS2_PLACEMENT_3D('',#208721,#124671,#124672);
#104264=AXIS2_PLACEMENT_3D('',#208722,#124673,#124674);
#104265=AXIS2_PLACEMENT_3D('',#208723,#124675,#124676);
#104266=AXIS2_PLACEMENT_3D('',#208742,#124677,#124678);
#104267=AXIS2_PLACEMENT_3D('',#208743,#124679,#124680);
#104268=AXIS2_PLACEMENT_3D('',#208744,#124681,#124682);
#104269=AXIS2_PLACEMENT_3D('',#208745,#124683,#124684);
#104270=AXIS2_PLACEMENT_3D('',#208746,#124685,#124686);
#104271=AXIS2_PLACEMENT_3D('',#208759,#124687,#124688);
#104272=AXIS2_PLACEMENT_3D('',#208772,#124689,#124690);
#104273=AXIS2_PLACEMENT_3D('',#208773,#124691,#124692);
#104274=AXIS2_PLACEMENT_3D('',#208774,#124693,#124694);
#104275=AXIS2_PLACEMENT_3D('',#208775,#124695,#124696);
#104276=AXIS2_PLACEMENT_3D('',#208776,#124697,#124698);
#104277=AXIS2_PLACEMENT_3D('',#208789,#124699,#124700);
#104278=AXIS2_PLACEMENT_3D('',#208790,#124701,#124702);
#104279=AXIS2_PLACEMENT_3D('',#208791,#124703,#124704);
#104280=AXIS2_PLACEMENT_3D('',#208792,#124705,#124706);
#104281=AXIS2_PLACEMENT_3D('',#208793,#124707,#124708);
#104282=AXIS2_PLACEMENT_3D('',#208806,#124709,#124710);
#104283=AXIS2_PLACEMENT_3D('',#208807,#124711,#124712);
#104284=AXIS2_PLACEMENT_3D('',#208808,#124713,#124714);
#104285=AXIS2_PLACEMENT_3D('',#208809,#124715,#124716);
#104286=AXIS2_PLACEMENT_3D('',#208810,#124717,#124718);
#104287=AXIS2_PLACEMENT_3D('',#208823,#124719,#124720);
#104288=AXIS2_PLACEMENT_3D('',#208836,#124721,#124722);
#104289=AXIS2_PLACEMENT_3D('',#208837,#124723,#124724);
#104290=AXIS2_PLACEMENT_3D('',#208838,#124725,#124726);
#104291=AXIS2_PLACEMENT_3D('',#208839,#124727,#124728);
#104292=AXIS2_PLACEMENT_3D('',#208840,#124729,#124730);
#104293=AXIS2_PLACEMENT_3D('',#208859,#124731,#124732);
#104294=AXIS2_PLACEMENT_3D('',#208860,#124733,#124734);
#104295=AXIS2_PLACEMENT_3D('',#208861,#124735,#124736);
#104296=AXIS2_PLACEMENT_3D('',#208862,#124737,#124738);
#104297=AXIS2_PLACEMENT_3D('',#208863,#124739,#124740);
#104298=AXIS2_PLACEMENT_3D('',#208876,#124741,#124742);
#104299=AXIS2_PLACEMENT_3D('',#208895,#124743,#124744);
#104300=AXIS2_PLACEMENT_3D('',#208896,#124745,#124746);
#104301=AXIS2_PLACEMENT_3D('',#208897,#124747,#124748);
#104302=AXIS2_PLACEMENT_3D('',#208898,#124749,#124750);
#104303=AXIS2_PLACEMENT_3D('',#208899,#124751,#124752);
#104304=AXIS2_PLACEMENT_3D('',#208918,#124753,#124754);
#104305=AXIS2_PLACEMENT_3D('',#208931,#124755,#124756);
#104306=AXIS2_PLACEMENT_3D('',#208932,#124757,#124758);
#104307=AXIS2_PLACEMENT_3D('',#208933,#124759,#124760);
#104308=AXIS2_PLACEMENT_3D('',#208934,#124761,#124762);
#104309=AXIS2_PLACEMENT_3D('',#208935,#124763,#124764);
#104310=AXIS2_PLACEMENT_3D('',#208954,#124765,#124766);
#104311=AXIS2_PLACEMENT_3D('',#208955,#124767,#124768);
#104312=AXIS2_PLACEMENT_3D('',#208956,#124769,#124770);
#104313=AXIS2_PLACEMENT_3D('',#208957,#124771,#124772);
#104314=AXIS2_PLACEMENT_3D('',#208958,#124773,#124774);
#104315=AXIS2_PLACEMENT_3D('',#208971,#124775,#124776);
#104316=AXIS2_PLACEMENT_3D('',#208984,#124777,#124778);
#104317=AXIS2_PLACEMENT_3D('',#208985,#124779,#124780);
#104318=AXIS2_PLACEMENT_3D('',#208986,#124781,#124782);
#104319=AXIS2_PLACEMENT_3D('',#208987,#124783,#124784);
#104320=AXIS2_PLACEMENT_3D('',#208988,#124785,#124786);
#104321=AXIS2_PLACEMENT_3D('',#209001,#124787,#124788);
#104322=AXIS2_PLACEMENT_3D('',#209002,#124789,#124790);
#104323=AXIS2_PLACEMENT_3D('',#209003,#124791,#124792);
#104324=AXIS2_PLACEMENT_3D('',#209004,#124793,#124794);
#104325=AXIS2_PLACEMENT_3D('',#209005,#124795,#124796);
#104326=AXIS2_PLACEMENT_3D('',#209018,#124797,#124798);
#104327=AXIS2_PLACEMENT_3D('',#209019,#124799,#124800);
#104328=AXIS2_PLACEMENT_3D('',#209020,#124801,#124802);
#104329=AXIS2_PLACEMENT_3D('',#209021,#124803,#124804);
#104330=AXIS2_PLACEMENT_3D('',#209022,#124805,#124806);
#104331=AXIS2_PLACEMENT_3D('',#209035,#124807,#124808);
#104332=AXIS2_PLACEMENT_3D('',#209048,#124809,#124810);
#104333=AXIS2_PLACEMENT_3D('',#209049,#124811,#124812);
#104334=AXIS2_PLACEMENT_3D('',#209050,#124813,#124814);
#104335=AXIS2_PLACEMENT_3D('',#209051,#124815,#124816);
#104336=AXIS2_PLACEMENT_3D('',#209052,#124817,#124818);
#104337=AXIS2_PLACEMENT_3D('',#209071,#124819,#124820);
#104338=AXIS2_PLACEMENT_3D('',#209072,#124821,#124822);
#104339=AXIS2_PLACEMENT_3D('',#209073,#124823,#124824);
#104340=AXIS2_PLACEMENT_3D('',#209074,#124825,#124826);
#104341=AXIS2_PLACEMENT_3D('',#209075,#124827,#124828);
#104342=AXIS2_PLACEMENT_3D('',#209088,#124829,#124830);
#104343=AXIS2_PLACEMENT_3D('',#209107,#124831,#124832);
#104344=AXIS2_PLACEMENT_3D('',#209108,#124833,#124834);
#104345=AXIS2_PLACEMENT_3D('',#209109,#124835,#124836);
#104346=AXIS2_PLACEMENT_3D('',#209110,#124837,#124838);
#104347=AXIS2_PLACEMENT_3D('',#209111,#124839,#124840);
#104348=AXIS2_PLACEMENT_3D('',#209130,#124841,#124842);
#104349=AXIS2_PLACEMENT_3D('',#209143,#124843,#124844);
#104350=AXIS2_PLACEMENT_3D('',#209144,#124845,#124846);
#104351=AXIS2_PLACEMENT_3D('',#209145,#124847,#124848);
#104352=AXIS2_PLACEMENT_3D('',#209146,#124849,#124850);
#104353=AXIS2_PLACEMENT_3D('',#209147,#124851,#124852);
#104354=AXIS2_PLACEMENT_3D('',#209166,#124853,#124854);
#104355=AXIS2_PLACEMENT_3D('',#209167,#124855,#124856);
#104356=AXIS2_PLACEMENT_3D('',#209168,#124857,#124858);
#104357=AXIS2_PLACEMENT_3D('',#209169,#124859,#124860);
#104358=AXIS2_PLACEMENT_3D('',#209170,#124861,#124862);
#104359=AXIS2_PLACEMENT_3D('',#209183,#124863,#124864);
#104360=AXIS2_PLACEMENT_3D('',#209196,#124865,#124866);
#104361=AXIS2_PLACEMENT_3D('',#209197,#124867,#124868);
#104362=AXIS2_PLACEMENT_3D('',#209198,#124869,#124870);
#104363=AXIS2_PLACEMENT_3D('',#209199,#124871,#124872);
#104364=AXIS2_PLACEMENT_3D('',#209200,#124873,#124874);
#104365=AXIS2_PLACEMENT_3D('',#209213,#124875,#124876);
#104366=AXIS2_PLACEMENT_3D('',#209214,#124877,#124878);
#104367=AXIS2_PLACEMENT_3D('',#209215,#124879,#124880);
#104368=AXIS2_PLACEMENT_3D('',#209216,#124881,#124882);
#104369=AXIS2_PLACEMENT_3D('',#209217,#124883,#124884);
#104370=AXIS2_PLACEMENT_3D('',#209230,#124885,#124886);
#104371=AXIS2_PLACEMENT_3D('',#209231,#124887,#124888);
#104372=AXIS2_PLACEMENT_3D('',#209232,#124889,#124890);
#104373=AXIS2_PLACEMENT_3D('',#209233,#124891,#124892);
#104374=AXIS2_PLACEMENT_3D('',#209234,#124893,#124894);
#104375=AXIS2_PLACEMENT_3D('',#209247,#124895,#124896);
#104376=AXIS2_PLACEMENT_3D('',#209260,#124897,#124898);
#104377=AXIS2_PLACEMENT_3D('',#209261,#124899,#124900);
#104378=AXIS2_PLACEMENT_3D('',#209262,#124901,#124902);
#104379=AXIS2_PLACEMENT_3D('',#209263,#124903,#124904);
#104380=AXIS2_PLACEMENT_3D('',#209264,#124905,#124906);
#104381=AXIS2_PLACEMENT_3D('',#209283,#124907,#124908);
#104382=AXIS2_PLACEMENT_3D('',#209284,#124909,#124910);
#104383=AXIS2_PLACEMENT_3D('',#209285,#124911,#124912);
#104384=AXIS2_PLACEMENT_3D('',#209286,#124913,#124914);
#104385=AXIS2_PLACEMENT_3D('',#209287,#124915,#124916);
#104386=AXIS2_PLACEMENT_3D('',#209300,#124917,#124918);
#104387=AXIS2_PLACEMENT_3D('',#209319,#124919,#124920);
#104388=AXIS2_PLACEMENT_3D('',#209320,#124921,#124922);
#104389=AXIS2_PLACEMENT_3D('',#209321,#124923,#124924);
#104390=AXIS2_PLACEMENT_3D('',#209322,#124925,#124926);
#104391=AXIS2_PLACEMENT_3D('',#209323,#124927,#124928);
#104392=AXIS2_PLACEMENT_3D('',#209342,#124929,#124930);
#104393=AXIS2_PLACEMENT_3D('',#209355,#124931,#124932);
#104394=AXIS2_PLACEMENT_3D('',#209356,#124933,#124934);
#104395=AXIS2_PLACEMENT_3D('',#209357,#124935,#124936);
#104396=AXIS2_PLACEMENT_3D('',#209358,#124937,#124938);
#104397=AXIS2_PLACEMENT_3D('',#209359,#124939,#124940);
#104398=AXIS2_PLACEMENT_3D('',#209378,#124941,#124942);
#104399=AXIS2_PLACEMENT_3D('',#209379,#124943,#124944);
#104400=AXIS2_PLACEMENT_3D('',#209380,#124945,#124946);
#104401=AXIS2_PLACEMENT_3D('',#209381,#124947,#124948);
#104402=AXIS2_PLACEMENT_3D('',#209382,#124949,#124950);
#104403=AXIS2_PLACEMENT_3D('',#209395,#124951,#124952);
#104404=AXIS2_PLACEMENT_3D('',#209408,#124953,#124954);
#104405=AXIS2_PLACEMENT_3D('',#209409,#124955,#124956);
#104406=AXIS2_PLACEMENT_3D('',#209410,#124957,#124958);
#104407=AXIS2_PLACEMENT_3D('',#209411,#124959,#124960);
#104408=AXIS2_PLACEMENT_3D('',#209412,#124961,#124962);
#104409=AXIS2_PLACEMENT_3D('',#209425,#124963,#124964);
#104410=AXIS2_PLACEMENT_3D('',#209426,#124965,#124966);
#104411=AXIS2_PLACEMENT_3D('',#209427,#124967,#124968);
#104412=AXIS2_PLACEMENT_3D('',#209428,#124969,#124970);
#104413=AXIS2_PLACEMENT_3D('',#209429,#124971,#124972);
#104414=AXIS2_PLACEMENT_3D('',#209442,#124973,#124974);
#104415=AXIS2_PLACEMENT_3D('',#209443,#124975,#124976);
#104416=AXIS2_PLACEMENT_3D('',#209444,#124977,#124978);
#104417=AXIS2_PLACEMENT_3D('',#209445,#124979,#124980);
#104418=AXIS2_PLACEMENT_3D('',#209446,#124981,#124982);
#104419=AXIS2_PLACEMENT_3D('',#209459,#124983,#124984);
#104420=AXIS2_PLACEMENT_3D('',#209472,#124985,#124986);
#104421=AXIS2_PLACEMENT_3D('',#209473,#124987,#124988);
#104422=AXIS2_PLACEMENT_3D('',#209474,#124989,#124990);
#104423=AXIS2_PLACEMENT_3D('',#209475,#124991,#124992);
#104424=AXIS2_PLACEMENT_3D('',#209476,#124993,#124994);
#104425=AXIS2_PLACEMENT_3D('',#209495,#124995,#124996);
#104426=AXIS2_PLACEMENT_3D('',#209496,#124997,#124998);
#104427=AXIS2_PLACEMENT_3D('',#209497,#124999,#125000);
#104428=AXIS2_PLACEMENT_3D('',#209498,#125001,#125002);
#104429=AXIS2_PLACEMENT_3D('',#209499,#125003,#125004);
#104430=AXIS2_PLACEMENT_3D('',#209512,#125005,#125006);
#104431=AXIS2_PLACEMENT_3D('',#209531,#125007,#125008);
#104432=AXIS2_PLACEMENT_3D('',#209532,#125009,#125010);
#104433=AXIS2_PLACEMENT_3D('',#209533,#125011,#125012);
#104434=AXIS2_PLACEMENT_3D('',#209534,#125013,#125014);
#104435=AXIS2_PLACEMENT_3D('',#209535,#125015,#125016);
#104436=AXIS2_PLACEMENT_3D('',#209554,#125017,#125018);
#104437=AXIS2_PLACEMENT_3D('',#209567,#125019,#125020);
#104438=AXIS2_PLACEMENT_3D('',#209568,#125021,#125022);
#104439=AXIS2_PLACEMENT_3D('',#209569,#125023,#125024);
#104440=AXIS2_PLACEMENT_3D('',#209570,#125025,#125026);
#104441=AXIS2_PLACEMENT_3D('',#209571,#125027,#125028);
#104442=AXIS2_PLACEMENT_3D('',#209590,#125029,#125030);
#104443=AXIS2_PLACEMENT_3D('',#209591,#125031,#125032);
#104444=AXIS2_PLACEMENT_3D('',#209592,#125033,#125034);
#104445=AXIS2_PLACEMENT_3D('',#209593,#125035,#125036);
#104446=AXIS2_PLACEMENT_3D('',#209594,#125037,#125038);
#104447=AXIS2_PLACEMENT_3D('',#209607,#125039,#125040);
#104448=AXIS2_PLACEMENT_3D('',#209620,#125041,#125042);
#104449=AXIS2_PLACEMENT_3D('',#209621,#125043,#125044);
#104450=AXIS2_PLACEMENT_3D('',#209622,#125045,#125046);
#104451=AXIS2_PLACEMENT_3D('',#209623,#125047,#125048);
#104452=AXIS2_PLACEMENT_3D('',#209624,#125049,#125050);
#104453=AXIS2_PLACEMENT_3D('',#209637,#125051,#125052);
#104454=AXIS2_PLACEMENT_3D('',#209638,#125053,#125054);
#104455=AXIS2_PLACEMENT_3D('',#209639,#125055,#125056);
#104456=AXIS2_PLACEMENT_3D('',#209640,#125057,#125058);
#104457=AXIS2_PLACEMENT_3D('',#209641,#125059,#125060);
#104458=AXIS2_PLACEMENT_3D('',#209654,#125061,#125062);
#104459=AXIS2_PLACEMENT_3D('',#209655,#125063,#125064);
#104460=AXIS2_PLACEMENT_3D('',#209656,#125065,#125066);
#104461=AXIS2_PLACEMENT_3D('',#209657,#125067,#125068);
#104462=AXIS2_PLACEMENT_3D('',#209658,#125069,#125070);
#104463=AXIS2_PLACEMENT_3D('',#209671,#125071,#125072);
#104464=AXIS2_PLACEMENT_3D('',#209684,#125073,#125074);
#104465=AXIS2_PLACEMENT_3D('',#209685,#125075,#125076);
#104466=AXIS2_PLACEMENT_3D('',#209686,#125077,#125078);
#104467=AXIS2_PLACEMENT_3D('',#209687,#125079,#125080);
#104468=AXIS2_PLACEMENT_3D('',#209688,#125081,#125082);
#104469=AXIS2_PLACEMENT_3D('',#209707,#125083,#125084);
#104470=AXIS2_PLACEMENT_3D('',#209708,#125085,#125086);
#104471=AXIS2_PLACEMENT_3D('',#209709,#125087,#125088);
#104472=AXIS2_PLACEMENT_3D('',#209710,#125089,#125090);
#104473=AXIS2_PLACEMENT_3D('',#209711,#125091,#125092);
#104474=AXIS2_PLACEMENT_3D('',#209724,#125093,#125094);
#104475=AXIS2_PLACEMENT_3D('',#209743,#125095,#125096);
#104476=AXIS2_PLACEMENT_3D('',#209744,#125097,#125098);
#104477=AXIS2_PLACEMENT_3D('',#209745,#125099,#125100);
#104478=AXIS2_PLACEMENT_3D('',#209746,#125101,#125102);
#104479=AXIS2_PLACEMENT_3D('',#209747,#125103,#125104);
#104480=AXIS2_PLACEMENT_3D('',#209766,#125105,#125106);
#104481=AXIS2_PLACEMENT_3D('',#209779,#125107,#125108);
#104482=AXIS2_PLACEMENT_3D('',#209780,#125109,#125110);
#104483=AXIS2_PLACEMENT_3D('',#209781,#125111,#125112);
#104484=AXIS2_PLACEMENT_3D('',#209782,#125113,#125114);
#104485=AXIS2_PLACEMENT_3D('',#209783,#125115,#125116);
#104486=AXIS2_PLACEMENT_3D('',#209802,#125117,#125118);
#104487=AXIS2_PLACEMENT_3D('',#209803,#125119,#125120);
#104488=AXIS2_PLACEMENT_3D('',#209804,#125121,#125122);
#104489=AXIS2_PLACEMENT_3D('',#209805,#125123,#125124);
#104490=AXIS2_PLACEMENT_3D('',#209806,#125125,#125126);
#104491=AXIS2_PLACEMENT_3D('',#209819,#125127,#125128);
#104492=AXIS2_PLACEMENT_3D('',#209832,#125129,#125130);
#104493=AXIS2_PLACEMENT_3D('',#209833,#125131,#125132);
#104494=AXIS2_PLACEMENT_3D('',#209834,#125133,#125134);
#104495=AXIS2_PLACEMENT_3D('',#209835,#125135,#125136);
#104496=AXIS2_PLACEMENT_3D('',#209836,#125137,#125138);
#104497=AXIS2_PLACEMENT_3D('',#209849,#125139,#125140);
#104498=AXIS2_PLACEMENT_3D('',#209850,#125141,#125142);
#104499=AXIS2_PLACEMENT_3D('',#209851,#125143,#125144);
#104500=AXIS2_PLACEMENT_3D('',#209852,#125145,#125146);
#104501=AXIS2_PLACEMENT_3D('',#209853,#125147,#125148);
#104502=AXIS2_PLACEMENT_3D('',#209866,#125149,#125150);
#104503=AXIS2_PLACEMENT_3D('',#209867,#125151,#125152);
#104504=AXIS2_PLACEMENT_3D('',#209868,#125153,#125154);
#104505=AXIS2_PLACEMENT_3D('',#209869,#125155,#125156);
#104506=AXIS2_PLACEMENT_3D('',#209870,#125157,#125158);
#104507=AXIS2_PLACEMENT_3D('',#209883,#125159,#125160);
#104508=AXIS2_PLACEMENT_3D('',#209896,#125161,#125162);
#104509=AXIS2_PLACEMENT_3D('',#209897,#125163,#125164);
#104510=AXIS2_PLACEMENT_3D('',#209898,#125165,#125166);
#104511=AXIS2_PLACEMENT_3D('',#209899,#125167,#125168);
#104512=AXIS2_PLACEMENT_3D('',#209900,#125169,#125170);
#104513=AXIS2_PLACEMENT_3D('',#209919,#125171,#125172);
#104514=AXIS2_PLACEMENT_3D('',#209920,#125173,#125174);
#104515=AXIS2_PLACEMENT_3D('',#209921,#125175,#125176);
#104516=AXIS2_PLACEMENT_3D('',#209922,#125177,#125178);
#104517=AXIS2_PLACEMENT_3D('',#209923,#125179,#125180);
#104518=AXIS2_PLACEMENT_3D('',#209936,#125181,#125182);
#104519=AXIS2_PLACEMENT_3D('',#209955,#125183,#125184);
#104520=AXIS2_PLACEMENT_3D('',#209956,#125185,#125186);
#104521=AXIS2_PLACEMENT_3D('',#209957,#125187,#125188);
#104522=AXIS2_PLACEMENT_3D('',#209958,#125189,#125190);
#104523=AXIS2_PLACEMENT_3D('',#209959,#125191,#125192);
#104524=AXIS2_PLACEMENT_3D('',#209978,#125193,#125194);
#104525=AXIS2_PLACEMENT_3D('',#209991,#125195,#125196);
#104526=AXIS2_PLACEMENT_3D('',#209992,#125197,#125198);
#104527=AXIS2_PLACEMENT_3D('',#209993,#125199,#125200);
#104528=AXIS2_PLACEMENT_3D('',#209994,#125201,#125202);
#104529=AXIS2_PLACEMENT_3D('',#209995,#125203,#125204);
#104530=AXIS2_PLACEMENT_3D('',#210014,#125205,#125206);
#104531=AXIS2_PLACEMENT_3D('',#210015,#125207,#125208);
#104532=AXIS2_PLACEMENT_3D('',#210016,#125209,#125210);
#104533=AXIS2_PLACEMENT_3D('',#210017,#125211,#125212);
#104534=AXIS2_PLACEMENT_3D('',#210018,#125213,#125214);
#104535=AXIS2_PLACEMENT_3D('',#210031,#125215,#125216);
#104536=AXIS2_PLACEMENT_3D('',#210044,#125217,#125218);
#104537=AXIS2_PLACEMENT_3D('',#210045,#125219,#125220);
#104538=AXIS2_PLACEMENT_3D('',#210046,#125221,#125222);
#104539=AXIS2_PLACEMENT_3D('',#210047,#125223,#125224);
#104540=AXIS2_PLACEMENT_3D('',#210048,#125225,#125226);
#104541=AXIS2_PLACEMENT_3D('',#210061,#125227,#125228);
#104542=AXIS2_PLACEMENT_3D('',#210062,#125229,#125230);
#104543=AXIS2_PLACEMENT_3D('',#210063,#125231,#125232);
#104544=AXIS2_PLACEMENT_3D('',#210064,#125233,#125234);
#104545=AXIS2_PLACEMENT_3D('',#210065,#125235,#125236);
#104546=AXIS2_PLACEMENT_3D('',#210078,#125237,#125238);
#104547=AXIS2_PLACEMENT_3D('',#210079,#125239,#125240);
#104548=AXIS2_PLACEMENT_3D('',#210080,#125241,#125242);
#104549=AXIS2_PLACEMENT_3D('',#210081,#125243,#125244);
#104550=AXIS2_PLACEMENT_3D('',#210082,#125245,#125246);
#104551=AXIS2_PLACEMENT_3D('',#210095,#125247,#125248);
#104552=AXIS2_PLACEMENT_3D('',#210108,#125249,#125250);
#104553=AXIS2_PLACEMENT_3D('',#210109,#125251,#125252);
#104554=AXIS2_PLACEMENT_3D('',#210110,#125253,#125254);
#104555=AXIS2_PLACEMENT_3D('',#210111,#125255,#125256);
#104556=AXIS2_PLACEMENT_3D('',#210112,#125257,#125258);
#104557=AXIS2_PLACEMENT_3D('',#210131,#125259,#125260);
#104558=AXIS2_PLACEMENT_3D('',#210132,#125261,#125262);
#104559=AXIS2_PLACEMENT_3D('',#210133,#125263,#125264);
#104560=AXIS2_PLACEMENT_3D('',#210134,#125265,#125266);
#104561=AXIS2_PLACEMENT_3D('',#210135,#125267,#125268);
#104562=AXIS2_PLACEMENT_3D('',#210148,#125269,#125270);
#104563=AXIS2_PLACEMENT_3D('',#210167,#125271,#125272);
#104564=AXIS2_PLACEMENT_3D('',#210168,#125273,#125274);
#104565=AXIS2_PLACEMENT_3D('',#210169,#125275,#125276);
#104566=AXIS2_PLACEMENT_3D('',#210170,#125277,#125278);
#104567=AXIS2_PLACEMENT_3D('',#210171,#125279,#125280);
#104568=AXIS2_PLACEMENT_3D('',#210190,#125281,#125282);
#104569=AXIS2_PLACEMENT_3D('',#210203,#125283,#125284);
#104570=AXIS2_PLACEMENT_3D('',#210204,#125285,#125286);
#104571=AXIS2_PLACEMENT_3D('',#210205,#125287,#125288);
#104572=AXIS2_PLACEMENT_3D('',#210206,#125289,#125290);
#104573=AXIS2_PLACEMENT_3D('',#210207,#125291,#125292);
#104574=AXIS2_PLACEMENT_3D('',#210226,#125293,#125294);
#104575=AXIS2_PLACEMENT_3D('',#210227,#125295,#125296);
#104576=AXIS2_PLACEMENT_3D('',#210228,#125297,#125298);
#104577=AXIS2_PLACEMENT_3D('',#210229,#125299,#125300);
#104578=AXIS2_PLACEMENT_3D('',#210230,#125301,#125302);
#104579=AXIS2_PLACEMENT_3D('',#210243,#125303,#125304);
#104580=AXIS2_PLACEMENT_3D('',#210256,#125305,#125306);
#104581=AXIS2_PLACEMENT_3D('',#210257,#125307,#125308);
#104582=AXIS2_PLACEMENT_3D('',#210258,#125309,#125310);
#104583=AXIS2_PLACEMENT_3D('',#210259,#125311,#125312);
#104584=AXIS2_PLACEMENT_3D('',#210260,#125313,#125314);
#104585=AXIS2_PLACEMENT_3D('',#210273,#125315,#125316);
#104586=AXIS2_PLACEMENT_3D('',#210274,#125317,#125318);
#104587=AXIS2_PLACEMENT_3D('',#210275,#125319,#125320);
#104588=AXIS2_PLACEMENT_3D('',#210276,#125321,#125322);
#104589=AXIS2_PLACEMENT_3D('',#210277,#125323,#125324);
#104590=AXIS2_PLACEMENT_3D('',#210290,#125325,#125326);
#104591=AXIS2_PLACEMENT_3D('',#210291,#125327,#125328);
#104592=AXIS2_PLACEMENT_3D('',#210292,#125329,#125330);
#104593=AXIS2_PLACEMENT_3D('',#210293,#125331,#125332);
#104594=AXIS2_PLACEMENT_3D('',#210294,#125333,#125334);
#104595=AXIS2_PLACEMENT_3D('',#210307,#125335,#125336);
#104596=AXIS2_PLACEMENT_3D('',#210320,#125337,#125338);
#104597=AXIS2_PLACEMENT_3D('',#210321,#125339,#125340);
#104598=AXIS2_PLACEMENT_3D('',#210322,#125341,#125342);
#104599=AXIS2_PLACEMENT_3D('',#210323,#125343,#125344);
#104600=AXIS2_PLACEMENT_3D('',#210324,#125345,#125346);
#104601=AXIS2_PLACEMENT_3D('',#210343,#125347,#125348);
#104602=AXIS2_PLACEMENT_3D('',#210344,#125349,#125350);
#104603=AXIS2_PLACEMENT_3D('',#210345,#125351,#125352);
#104604=AXIS2_PLACEMENT_3D('',#210346,#125353,#125354);
#104605=AXIS2_PLACEMENT_3D('',#210347,#125355,#125356);
#104606=AXIS2_PLACEMENT_3D('',#210360,#125357,#125358);
#104607=AXIS2_PLACEMENT_3D('',#210379,#125359,#125360);
#104608=AXIS2_PLACEMENT_3D('',#210380,#125361,#125362);
#104609=AXIS2_PLACEMENT_3D('',#210381,#125363,#125364);
#104610=AXIS2_PLACEMENT_3D('',#210382,#125365,#125366);
#104611=AXIS2_PLACEMENT_3D('',#210383,#125367,#125368);
#104612=AXIS2_PLACEMENT_3D('',#210402,#125369,#125370);
#104613=AXIS2_PLACEMENT_3D('',#210415,#125371,#125372);
#104614=AXIS2_PLACEMENT_3D('',#210416,#125373,#125374);
#104615=AXIS2_PLACEMENT_3D('',#210417,#125375,#125376);
#104616=AXIS2_PLACEMENT_3D('',#210418,#125377,#125378);
#104617=AXIS2_PLACEMENT_3D('',#210419,#125379,#125380);
#104618=AXIS2_PLACEMENT_3D('',#210438,#125381,#125382);
#104619=AXIS2_PLACEMENT_3D('',#210439,#125383,#125384);
#104620=AXIS2_PLACEMENT_3D('',#210440,#125385,#125386);
#104621=AXIS2_PLACEMENT_3D('',#210441,#125387,#125388);
#104622=AXIS2_PLACEMENT_3D('',#210442,#125389,#125390);
#104623=AXIS2_PLACEMENT_3D('',#210455,#125391,#125392);
#104624=AXIS2_PLACEMENT_3D('',#210468,#125393,#125394);
#104625=AXIS2_PLACEMENT_3D('',#210469,#125395,#125396);
#104626=AXIS2_PLACEMENT_3D('',#210470,#125397,#125398);
#104627=AXIS2_PLACEMENT_3D('',#210471,#125399,#125400);
#104628=AXIS2_PLACEMENT_3D('',#210472,#125401,#125402);
#104629=AXIS2_PLACEMENT_3D('',#210485,#125403,#125404);
#104630=AXIS2_PLACEMENT_3D('',#210486,#125405,#125406);
#104631=AXIS2_PLACEMENT_3D('',#210487,#125407,#125408);
#104632=AXIS2_PLACEMENT_3D('',#210490,#125409,#125410);
#104633=AXIS2_PLACEMENT_3D('',#210492,#125411,#125412);
#104634=AXIS2_PLACEMENT_3D('',#210494,#125413,#125414);
#104635=AXIS2_PLACEMENT_3D('',#210495,#125415,#125416);
#104636=AXIS2_PLACEMENT_3D('',#210496,#125417,#125418);
#104637=AXIS2_PLACEMENT_3D('',#210499,#125419,#125420);
#104638=AXIS2_PLACEMENT_3D('',#210501,#125421,#125422);
#104639=AXIS2_PLACEMENT_3D('',#210503,#125423,#125424);
#104640=AXIS2_PLACEMENT_3D('',#210504,#125425,#125426);
#104641=AXIS2_PLACEMENT_3D('',#210505,#125427,#125428);
#104642=AXIS2_PLACEMENT_3D('',#210508,#125429,#125430);
#104643=AXIS2_PLACEMENT_3D('',#210510,#125431,#125432);
#104644=AXIS2_PLACEMENT_3D('',#210512,#125433,#125434);
#104645=AXIS2_PLACEMENT_3D('',#210513,#125435,#125436);
#104646=AXIS2_PLACEMENT_3D('',#210514,#125437,#125438);
#104647=AXIS2_PLACEMENT_3D('',#210517,#125439,#125440);
#104648=AXIS2_PLACEMENT_3D('',#210519,#125441,#125442);
#104649=AXIS2_PLACEMENT_3D('',#210521,#125443,#125444);
#104650=AXIS2_PLACEMENT_3D('',#210523,#125445,#125446);
#104651=AXIS2_PLACEMENT_3D('',#210524,#125447,#125448);
#104652=AXIS2_PLACEMENT_3D('',#210525,#125449,#125450);
#104653=AXIS2_PLACEMENT_3D('',#210527,#125451,#125452);
#104654=AXIS2_PLACEMENT_3D('',#210529,#125453,#125454);
#104655=AXIS2_PLACEMENT_3D('',#210531,#125455,#125456);
#104656=AXIS2_PLACEMENT_3D('',#210532,#125457,#125458);
#104657=AXIS2_PLACEMENT_3D('',#210533,#125459,#125460);
#104658=AXIS2_PLACEMENT_3D('',#210535,#125461,#125462);
#104659=AXIS2_PLACEMENT_3D('',#210537,#125463,#125464);
#104660=AXIS2_PLACEMENT_3D('',#210538,#125465,#125466);
#104661=AXIS2_PLACEMENT_3D('',#210539,#125467,#125468);
#104662=AXIS2_PLACEMENT_3D('',#210541,#125469,#125470);
#104663=AXIS2_PLACEMENT_3D('',#210543,#125471,#125472);
#104664=AXIS2_PLACEMENT_3D('',#210545,#125473,#125474);
#104665=AXIS2_PLACEMENT_3D('',#210546,#125475,#125476);
#104666=AXIS2_PLACEMENT_3D('',#210547,#125477,#125478);
#104667=AXIS2_PLACEMENT_3D('',#210549,#125479,#125480);
#104668=AXIS2_PLACEMENT_3D('',#210551,#125481,#125482);
#104669=AXIS2_PLACEMENT_3D('',#210552,#125483,#125484);
#104670=AXIS2_PLACEMENT_3D('',#210553,#125485,#125486);
#104671=AXIS2_PLACEMENT_3D('',#210555,#125487,#125488);
#104672=AXIS2_PLACEMENT_3D('',#210558,#125490,#125491);
#104673=AXIS2_PLACEMENT_3D('',#210559,#125492,#125493);
#104674=AXIS2_PLACEMENT_3D('',#210561,#125495,#125496);
#104675=AXIS2_PLACEMENT_3D('',#210564,#125497,#125498);
#104676=AXIS2_PLACEMENT_3D('',#210612,#125500,#125501);
#104677=AXIS2_PLACEMENT_3D('',#210657,#125503,#125504);
#104678=AXIS2_PLACEMENT_3D('',#210705,#125506,#125507);
#104679=AXIS2_PLACEMENT_3D('',#210750,#125509,#125510);
#104680=AXIS2_PLACEMENT_3D('',#210798,#125512,#125513);
#104681=AXIS2_PLACEMENT_3D('',#210843,#125515,#125516);
#104682=AXIS2_PLACEMENT_3D('',#210891,#125518,#125519);
#104683=AXIS2_PLACEMENT_3D('',#210936,#125521,#125522);
#104684=AXIS2_PLACEMENT_3D('',#210984,#125524,#125525);
#104685=AXIS2_PLACEMENT_3D('',#211029,#125527,#125528);
#104686=AXIS2_PLACEMENT_3D('',#211077,#125530,#125531);
#104687=AXIS2_PLACEMENT_3D('',#211122,#125533,#125534);
#104688=AXIS2_PLACEMENT_3D('',#211170,#125536,#125537);
#104689=AXIS2_PLACEMENT_3D('',#211215,#125539,#125540);
#104690=AXIS2_PLACEMENT_3D('',#211263,#125542,#125543);
#104691=AXIS2_PLACEMENT_3D('',#211308,#125545,#125546);
#104692=AXIS2_PLACEMENT_3D('',#211356,#125548,#125549);
#104693=AXIS2_PLACEMENT_3D('',#211401,#125551,#125552);
#104694=AXIS2_PLACEMENT_3D('',#211449,#125554,#125555);
#104695=AXIS2_PLACEMENT_3D('',#211494,#125557,#125558);
#104696=AXIS2_PLACEMENT_3D('',#211542,#125560,#125561);
#104697=AXIS2_PLACEMENT_3D('',#211587,#125563,#125564);
#104698=AXIS2_PLACEMENT_3D('',#211635,#125566,#125567);
#104699=AXIS2_PLACEMENT_3D('',#211680,#125569,#125570);
#104700=AXIS2_PLACEMENT_3D('',#211728,#125572,#125573);
#104701=AXIS2_PLACEMENT_3D('',#211773,#125575,#125576);
#104702=AXIS2_PLACEMENT_3D('',#211821,#125578,#125579);
#104703=AXIS2_PLACEMENT_3D('',#211866,#125581,#125582);
#104704=AXIS2_PLACEMENT_3D('',#211914,#125584,#125585);
#104705=AXIS2_PLACEMENT_3D('',#211959,#125587,#125588);
#104706=AXIS2_PLACEMENT_3D('',#212007,#125590,#125591);
#104707=AXIS2_PLACEMENT_3D('',#212052,#125593,#125594);
#104708=AXIS2_PLACEMENT_3D('',#212100,#125596,#125597);
#104709=AXIS2_PLACEMENT_3D('',#212145,#125599,#125600);
#104710=AXIS2_PLACEMENT_3D('',#212193,#125602,#125603);
#104711=AXIS2_PLACEMENT_3D('',#212238,#125605,#125606);
#104712=AXIS2_PLACEMENT_3D('',#212286,#125608,#125609);
#104713=AXIS2_PLACEMENT_3D('',#212331,#125611,#125612);
#104714=AXIS2_PLACEMENT_3D('',#212379,#125614,#125615);
#104715=AXIS2_PLACEMENT_3D('',#212424,#125617,#125618);
#104716=AXIS2_PLACEMENT_3D('',#212472,#125620,#125621);
#104717=AXIS2_PLACEMENT_3D('',#212517,#125623,#125624);
#104718=AXIS2_PLACEMENT_3D('',#212565,#125626,#125627);
#104719=AXIS2_PLACEMENT_3D('',#212610,#125629,#125630);
#104720=AXIS2_PLACEMENT_3D('',#212658,#125632,#125633);
#104721=AXIS2_PLACEMENT_3D('',#212703,#125635,#125636);
#104722=AXIS2_PLACEMENT_3D('',#212751,#125638,#125639);
#104723=AXIS2_PLACEMENT_3D('',#212796,#125641,#125642);
#104724=AXIS2_PLACEMENT_3D('',#212844,#125644,#125645);
#104725=AXIS2_PLACEMENT_3D('',#212889,#125647,#125648);
#104726=AXIS2_PLACEMENT_3D('',#212937,#125650,#125651);
#104727=AXIS2_PLACEMENT_3D('',#212982,#125653,#125654);
#104728=AXIS2_PLACEMENT_3D('',#213030,#125656,#125657);
#104729=AXIS2_PLACEMENT_3D('',#213075,#125659,#125660);
#104730=AXIS2_PLACEMENT_3D('',#213123,#125662,#125663);
#104731=AXIS2_PLACEMENT_3D('',#213168,#125665,#125666);
#104732=AXIS2_PLACEMENT_3D('',#213216,#125668,#125669);
#104733=AXIS2_PLACEMENT_3D('',#213261,#125671,#125672);
#104734=AXIS2_PLACEMENT_3D('',#213309,#125674,#125675);
#104735=AXIS2_PLACEMENT_3D('',#213400,#125679,#125680);
#104736=AXIS2_PLACEMENT_3D('',#213445,#125682,#125683);
#104737=AXIS2_PLACEMENT_3D('',#213493,#125685,#125686);
#104738=AXIS2_PLACEMENT_3D('',#213538,#125688,#125689);
#104739=AXIS2_PLACEMENT_3D('',#213586,#125691,#125692);
#104740=AXIS2_PLACEMENT_3D('',#213631,#125694,#125695);
#104741=AXIS2_PLACEMENT_3D('',#213679,#125697,#125698);
#104742=AXIS2_PLACEMENT_3D('',#213724,#125700,#125701);
#104743=AXIS2_PLACEMENT_3D('',#213772,#125703,#125704);
#104744=AXIS2_PLACEMENT_3D('',#213817,#125706,#125707);
#104745=AXIS2_PLACEMENT_3D('',#213865,#125709,#125710);
#104746=AXIS2_PLACEMENT_3D('',#213910,#125712,#125713);
#104747=AXIS2_PLACEMENT_3D('',#213958,#125715,#125716);
#104748=AXIS2_PLACEMENT_3D('',#214003,#125718,#125719);
#104749=AXIS2_PLACEMENT_3D('',#214051,#125721,#125722);
#104750=AXIS2_PLACEMENT_3D('',#214096,#125724,#125725);
#104751=AXIS2_PLACEMENT_3D('',#214144,#125727,#125728);
#104752=AXIS2_PLACEMENT_3D('',#214189,#125730,#125731);
#104753=AXIS2_PLACEMENT_3D('',#214237,#125733,#125734);
#104754=AXIS2_PLACEMENT_3D('',#214282,#125736,#125737);
#104755=AXIS2_PLACEMENT_3D('',#214330,#125739,#125740);
#104756=AXIS2_PLACEMENT_3D('',#214375,#125742,#125743);
#104757=AXIS2_PLACEMENT_3D('',#214423,#125745,#125746);
#104758=AXIS2_PLACEMENT_3D('',#214468,#125748,#125749);
#104759=AXIS2_PLACEMENT_3D('',#214516,#125751,#125752);
#104760=AXIS2_PLACEMENT_3D('',#214561,#125754,#125755);
#104761=AXIS2_PLACEMENT_3D('',#214609,#125757,#125758);
#104762=AXIS2_PLACEMENT_3D('',#214654,#125760,#125761);
#104763=AXIS2_PLACEMENT_3D('',#214702,#125763,#125764);
#104764=AXIS2_PLACEMENT_3D('',#214792,#125767,#125768);
#104765=AXIS2_PLACEMENT_3D('',#214837,#125770,#125771);
#104766=AXIS2_PLACEMENT_3D('',#214885,#125773,#125774);
#104767=AXIS2_PLACEMENT_3D('',#214930,#125776,#125777);
#104768=AXIS2_PLACEMENT_3D('',#214978,#125779,#125780);
#104769=AXIS2_PLACEMENT_3D('',#215023,#125782,#125783);
#104770=AXIS2_PLACEMENT_3D('',#215071,#125785,#125786);
#104771=AXIS2_PLACEMENT_3D('',#215116,#125788,#125789);
#104772=AXIS2_PLACEMENT_3D('',#215164,#125791,#125792);
#104773=AXIS2_PLACEMENT_3D('',#215209,#125794,#125795);
#104774=AXIS2_PLACEMENT_3D('',#215257,#125797,#125798);
#104775=AXIS2_PLACEMENT_3D('',#215302,#125800,#125801);
#104776=AXIS2_PLACEMENT_3D('',#215350,#125803,#125804);
#104777=AXIS2_PLACEMENT_3D('',#215395,#125806,#125807);
#104778=AXIS2_PLACEMENT_3D('',#215443,#125809,#125810);
#104779=AXIS2_PLACEMENT_3D('',#215488,#125812,#125813);
#104780=AXIS2_PLACEMENT_3D('',#215536,#125815,#125816);
#104781=AXIS2_PLACEMENT_3D('',#215581,#125818,#125819);
#104782=AXIS2_PLACEMENT_3D('',#215629,#125821,#125822);
#104783=AXIS2_PLACEMENT_3D('',#215674,#125824,#125825);
#104784=AXIS2_PLACEMENT_3D('',#215722,#125827,#125828);
#104785=AXIS2_PLACEMENT_3D('',#215767,#125830,#125831);
#104786=AXIS2_PLACEMENT_3D('',#215815,#125833,#125834);
#104787=AXIS2_PLACEMENT_3D('',#215860,#125836,#125837);
#104788=AXIS2_PLACEMENT_3D('',#215908,#125839,#125840);
#104789=AXIS2_PLACEMENT_3D('',#215953,#125842,#125843);
#104790=AXIS2_PLACEMENT_3D('',#216001,#125845,#125846);
#104791=AXIS2_PLACEMENT_3D('',#216046,#125848,#125849);
#104792=AXIS2_PLACEMENT_3D('',#216094,#125851,#125852);
#104793=AXIS2_PLACEMENT_3D('',#216137,#125854,#125855);
#104794=AXIS2_PLACEMENT_3D('',#216179,#125857,#125858);
#104795=AXIS2_PLACEMENT_3D('',#216224,#125860,#125861);
#104796=AXIS2_PLACEMENT_3D('',#216266,#125863,#125864);
#104797=AXIS2_PLACEMENT_3D('',#216311,#125866,#125867);
#104798=AXIS2_PLACEMENT_3D('',#216353,#125869,#125870);
#104799=AXIS2_PLACEMENT_3D('',#216398,#125872,#125873);
#104800=AXIS2_PLACEMENT_3D('',#216440,#125875,#125876);
#104801=AXIS2_PLACEMENT_3D('',#216485,#125878,#125879);
#104802=AXIS2_PLACEMENT_3D('',#216527,#125881,#125882);
#104803=AXIS2_PLACEMENT_3D('',#216572,#125884,#125885);
#104804=AXIS2_PLACEMENT_3D('',#216614,#125887,#125888);
#104805=AXIS2_PLACEMENT_3D('',#216659,#125890,#125891);
#104806=AXIS2_PLACEMENT_3D('',#216701,#125893,#125894);
#104807=AXIS2_PLACEMENT_3D('',#216746,#125896,#125897);
#104808=AXIS2_PLACEMENT_3D('',#216788,#125899,#125900);
#104809=AXIS2_PLACEMENT_3D('',#216833,#125902,#125903);
#104810=AXIS2_PLACEMENT_3D('',#216875,#125905,#125906);
#104811=AXIS2_PLACEMENT_3D('',#216920,#125908,#125909);
#104812=AXIS2_PLACEMENT_3D('',#216962,#125911,#125912);
#104813=AXIS2_PLACEMENT_3D('',#217007,#125914,#125915);
#104814=AXIS2_PLACEMENT_3D('',#217049,#125917,#125918);
#104815=AXIS2_PLACEMENT_3D('',#217094,#125920,#125921);
#104816=AXIS2_PLACEMENT_3D('',#217136,#125923,#125924);
#104817=AXIS2_PLACEMENT_3D('',#217181,#125926,#125927);
#104818=AXIS2_PLACEMENT_3D('',#217223,#125929,#125930);
#104819=AXIS2_PLACEMENT_3D('',#217268,#125932,#125933);
#104820=AXIS2_PLACEMENT_3D('',#217310,#125935,#125936);
#104821=AXIS2_PLACEMENT_3D('',#217355,#125938,#125939);
#104822=AXIS2_PLACEMENT_3D('',#217397,#125941,#125942);
#104823=AXIS2_PLACEMENT_3D('',#217442,#125944,#125945);
#104824=AXIS2_PLACEMENT_3D('',#217484,#125947,#125948);
#104825=AXIS2_PLACEMENT_3D('',#217529,#125950,#125951);
#104826=AXIS2_PLACEMENT_3D('',#217571,#125953,#125954);
#104827=AXIS2_PLACEMENT_3D('',#217616,#125956,#125957);
#104828=AXIS2_PLACEMENT_3D('',#217658,#125959,#125960);
#104829=AXIS2_PLACEMENT_3D('',#217703,#125962,#125963);
#104830=AXIS2_PLACEMENT_3D('',#217745,#125965,#125966);
#104831=AXIS2_PLACEMENT_3D('',#217790,#125968,#125969);
#104832=AXIS2_PLACEMENT_3D('',#217832,#125971,#125972);
#104833=AXIS2_PLACEMENT_3D('',#217877,#125974,#125975);
#104834=AXIS2_PLACEMENT_3D('',#217919,#125977,#125978);
#104835=AXIS2_PLACEMENT_3D('',#217964,#125980,#125981);
#104836=AXIS2_PLACEMENT_3D('',#218006,#125983,#125984);
#104837=AXIS2_PLACEMENT_3D('',#218051,#125986,#125987);
#104838=AXIS2_PLACEMENT_3D('',#218093,#125989,#125990);
#104839=AXIS2_PLACEMENT_3D('',#218138,#125992,#125993);
#104840=AXIS2_PLACEMENT_3D('',#218180,#125995,#125996);
#104841=AXIS2_PLACEMENT_3D('',#218225,#125998,#125999);
#104842=AXIS2_PLACEMENT_3D('',#218267,#126001,#126002);
#104843=AXIS2_PLACEMENT_3D('',#218312,#126004,#126005);
#104844=AXIS2_PLACEMENT_3D('',#218354,#126007,#126008);
#104845=AXIS2_PLACEMENT_3D('',#218399,#126010,#126011);
#104846=AXIS2_PLACEMENT_3D('',#218441,#126013,#126014);
#104847=AXIS2_PLACEMENT_3D('',#218486,#126016,#126017);
#104848=AXIS2_PLACEMENT_3D('',#218528,#126019,#126020);
#104849=AXIS2_PLACEMENT_3D('',#218573,#126022,#126023);
#104850=AXIS2_PLACEMENT_3D('',#218615,#126025,#126026);
#104851=AXIS2_PLACEMENT_3D('',#218660,#126028,#126029);
#104852=AXIS2_PLACEMENT_3D('',#218702,#126031,#126032);
#104853=AXIS2_PLACEMENT_3D('',#218747,#126034,#126035);
#104854=AXIS2_PLACEMENT_3D('',#218750,#126037,#126038);
#104855=AXIS2_PLACEMENT_3D('',#218792,#126040,#126041);
#104856=AXIS2_PLACEMENT_3D('',#218837,#126043,#126044);
#104857=AXIS2_PLACEMENT_3D('',#218879,#126046,#126047);
#104858=AXIS2_PLACEMENT_3D('',#218924,#126049,#126050);
#104859=AXIS2_PLACEMENT_3D('',#218966,#126052,#126053);
#104860=AXIS2_PLACEMENT_3D('',#219011,#126055,#126056);
#104861=AXIS2_PLACEMENT_3D('',#219053,#126058,#126059);
#104862=AXIS2_PLACEMENT_3D('',#219098,#126061,#126062);
#104863=AXIS2_PLACEMENT_3D('',#219140,#126064,#126065);
#104864=AXIS2_PLACEMENT_3D('',#219185,#126067,#126068);
#104865=AXIS2_PLACEMENT_3D('',#219227,#126070,#126071);
#104866=AXIS2_PLACEMENT_3D('',#219272,#126073,#126074);
#104867=AXIS2_PLACEMENT_3D('',#219314,#126076,#126077);
#104868=AXIS2_PLACEMENT_3D('',#219359,#126079,#126080);
#104869=AXIS2_PLACEMENT_3D('',#219401,#126082,#126083);
#104870=AXIS2_PLACEMENT_3D('',#219446,#126085,#126086);
#104871=AXIS2_PLACEMENT_3D('',#219488,#126088,#126089);
#104872=AXIS2_PLACEMENT_3D('',#219533,#126091,#126092);
#104873=AXIS2_PLACEMENT_3D('',#219575,#126094,#126095);
#104874=AXIS2_PLACEMENT_3D('',#219620,#126097,#126098);
#104875=AXIS2_PLACEMENT_3D('',#219662,#126100,#126101);
#104876=AXIS2_PLACEMENT_3D('',#219707,#126103,#126104);
#104877=AXIS2_PLACEMENT_3D('',#219749,#126106,#126107);
#104878=AXIS2_PLACEMENT_3D('',#219794,#126109,#126110);
#104879=AXIS2_PLACEMENT_3D('',#219836,#126112,#126113);
#104880=AXIS2_PLACEMENT_3D('',#219881,#126115,#126116);
#104881=AXIS2_PLACEMENT_3D('',#219923,#126118,#126119);
#104882=AXIS2_PLACEMENT_3D('',#219968,#126121,#126122);
#104883=AXIS2_PLACEMENT_3D('',#220010,#126124,#126125);
#104884=AXIS2_PLACEMENT_3D('',#220094,#126128,#126129);
#104885=AXIS2_PLACEMENT_3D('',#220139,#126131,#126132);
#104886=AXIS2_PLACEMENT_3D('',#220181,#126134,#126135);
#104887=AXIS2_PLACEMENT_3D('',#220226,#126137,#126138);
#104888=AXIS2_PLACEMENT_3D('',#220268,#126140,#126141);
#104889=AXIS2_PLACEMENT_3D('',#220313,#126143,#126144);
#104890=AXIS2_PLACEMENT_3D('',#220355,#126146,#126147);
#104891=AXIS2_PLACEMENT_3D('',#220400,#126149,#126150);
#104892=AXIS2_PLACEMENT_3D('',#220442,#126152,#126153);
#104893=AXIS2_PLACEMENT_3D('',#220487,#126155,#126156);
#104894=AXIS2_PLACEMENT_3D('',#220529,#126158,#126159);
#104895=AXIS2_PLACEMENT_3D('',#220574,#126161,#126162);
#104896=AXIS2_PLACEMENT_3D('',#220616,#126164,#126165);
#104897=AXIS2_PLACEMENT_3D('',#220661,#126167,#126168);
#104898=AXIS2_PLACEMENT_3D('',#220703,#126170,#126171);
#104899=AXIS2_PLACEMENT_3D('',#220748,#126173,#126174);
#104900=AXIS2_PLACEMENT_3D('',#220790,#126176,#126177);
#104901=AXIS2_PLACEMENT_3D('',#220835,#126179,#126180);
#104902=AXIS2_PLACEMENT_3D('',#220877,#126182,#126183);
#104903=AXIS2_PLACEMENT_3D('',#220922,#126185,#126186);
#104904=AXIS2_PLACEMENT_3D('',#220964,#126188,#126189);
#104905=AXIS2_PLACEMENT_3D('',#221009,#126191,#126192);
#104906=AXIS2_PLACEMENT_3D('',#221051,#126194,#126195);
#104907=AXIS2_PLACEMENT_3D('',#221096,#126197,#126198);
#104908=AXIS2_PLACEMENT_3D('',#221138,#126200,#126201);
#104909=AXIS2_PLACEMENT_3D('',#221183,#126203,#126204);
#104910=AXIS2_PLACEMENT_3D('',#221225,#126206,#126207);
#104911=AXIS2_PLACEMENT_3D('',#221270,#126209,#126210);
#104912=AXIS2_PLACEMENT_3D('',#221312,#126212,#126213);
#104913=AXIS2_PLACEMENT_3D('',#221355,#126215,#126216);
#104914=AXIS2_PLACEMENT_3D('',#221358,#126217,#126218);
#104915=AXIS2_PLACEMENT_3D('',#221360,#126220,#126221);
#104916=AXIS2_PLACEMENT_3D('',#221361,#126222,#126223);
#104917=AXIS2_PLACEMENT_3D('',#221364,#126225,#126226);
#104918=AXIS2_PLACEMENT_3D('',#221365,#126227,#126228);
#104919=AXIS2_PLACEMENT_3D('',#221368,#126229,#126230);
#104920=AXIS2_PLACEMENT_3D('',#221372,#126232,#126233);
#104921=AXIS2_PLACEMENT_3D('',#221376,#126235,#126236);
#104922=AXIS2_PLACEMENT_3D('',#221377,#126237,#126238);
#104923=AXIS2_PLACEMENT_3D('',#221378,#126239,#126240);
#104924=AXIS2_PLACEMENT_3D('',#221381,#126241,#126242);
#104925=AXIS2_PLACEMENT_3D('',#221384,#126245,#126246);
#104926=AXIS2_PLACEMENT_3D('',#221387,#126247,#126248);
#104927=AXIS2_PLACEMENT_3D('',#221391,#126250,#126251);
#104928=AXIS2_PLACEMENT_3D('',#221393,#126253,#126254);
#104929=AXIS2_PLACEMENT_3D('',#221396,#126255,#126256);
#104930=AXIS2_PLACEMENT_3D('',#221400,#126258,#126259);
#104931=AXIS2_PLACEMENT_3D('',#221404,#126261,#126262);
#104932=AXIS2_PLACEMENT_3D('',#221405,#126263,#126264);
#104933=AXIS2_PLACEMENT_3D('',#221406,#126265,#126266);
#104934=AXIS2_PLACEMENT_3D('',#221409,#126267,#126268);
#104935=AXIS2_PLACEMENT_3D('',#221412,#126271,#126272);
#104936=AXIS2_PLACEMENT_3D('',#221413,#126273,#126274);
#104937=AXIS2_PLACEMENT_3D('',#221414,#126275,#126276);
#104938=AXIS2_PLACEMENT_3D('',#221415,#126277,#126278);
#104939=AXIS2_PLACEMENT_3D('',#221416,#126279,#126280);
#104940=AXIS2_PLACEMENT_3D('',#221417,#126281,#126282);
#104941=AXIS2_PLACEMENT_3D('',#221418,#126283,#126284);
#104942=AXIS2_PLACEMENT_3D('',#221419,#126285,#126286);
#104943=AXIS2_PLACEMENT_3D('',#221420,#126287,#126288);
#104944=AXIS2_PLACEMENT_3D('',#221421,#126289,#126290);
#104945=AXIS2_PLACEMENT_3D('',#221422,#126291,#126292);
#104946=AXIS2_PLACEMENT_3D('',#221423,#126293,#126294);
#104947=AXIS2_PLACEMENT_3D('',#221424,#126295,#126296);
#104948=AXIS2_PLACEMENT_3D('',#221427,#126297,#126298);
#104949=AXIS2_PLACEMENT_3D('',#221431,#126300,#126301);
#104950=AXIS2_PLACEMENT_3D('',#221433,#126302,#126303);
#104951=AXIS2_PLACEMENT_3D('',#221435,#126304,#126305);
#104952=AXIS2_PLACEMENT_3D('',#221437,#126307,#126308);
#104953=AXIS2_PLACEMENT_3D('',#221441,#126310,#126311);
#104954=AXIS2_PLACEMENT_3D('',#221443,#126313,#126314);
#104955=AXIS2_PLACEMENT_3D('',#221446,#126315,#126316);
#104956=AXIS2_PLACEMENT_3D('',#221450,#126318,#126319);
#104957=AXIS2_PLACEMENT_3D('',#221452,#126321,#126322);
#104958=AXIS2_PLACEMENT_3D('',#221455,#126323,#126324);
#104959=AXIS2_PLACEMENT_3D('',#221459,#126326,#126327);
#104960=AXIS2_PLACEMENT_3D('',#221461,#126328,#126329);
#104961=AXIS2_PLACEMENT_3D('',#221463,#126330,#126331);
#104962=AXIS2_PLACEMENT_3D('',#221465,#126333,#126334);
#104963=AXIS2_PLACEMENT_3D('',#221469,#126336,#126337);
#104964=AXIS2_PLACEMENT_3D('',#221471,#126339,#126340);
#104965=AXIS2_PLACEMENT_3D('',#221472,#126341,#126342);
#104966=AXIS2_PLACEMENT_3D('',#221473,#126343,#126344);
#104967=AXIS2_PLACEMENT_3D('',#221474,#126345,#126346);
#104968=AXIS2_PLACEMENT_3D('',#221475,#126347,#126348);
#104969=AXIS2_PLACEMENT_3D('',#221476,#126349,#126350);
#104970=AXIS2_PLACEMENT_3D('',#221477,#126351,#126352);
#104971=AXIS2_PLACEMENT_3D('',#221478,#126353,#126354);
#104972=AXIS2_PLACEMENT_3D('',#221479,#126355,#126356);
#104973=AXIS2_PLACEMENT_3D('',#221480,#126357,#126358);
#104974=AXIS2_PLACEMENT_3D('',#221481,#126359,#126360);
#104975=AXIS2_PLACEMENT_3D('',#221482,#126361,#126362);
#104976=AXIS2_PLACEMENT_3D('',#221483,#126363,#126364);
#104977=AXIS2_PLACEMENT_3D('',#221486,#126365,#126366);
#104978=AXIS2_PLACEMENT_3D('',#221490,#126368,#126369);
#104979=AXIS2_PLACEMENT_3D('',#221492,#126370,#126371);
#104980=AXIS2_PLACEMENT_3D('',#221494,#126372,#126373);
#104981=AXIS2_PLACEMENT_3D('',#221496,#126375,#126376);
#104982=AXIS2_PLACEMENT_3D('',#221500,#126378,#126379);
#104983=AXIS2_PLACEMENT_3D('',#221502,#126381,#126382);
#104984=AXIS2_PLACEMENT_3D('',#221505,#126383,#126384);
#104985=AXIS2_PLACEMENT_3D('',#221509,#126386,#126387);
#104986=AXIS2_PLACEMENT_3D('',#221511,#126389,#126390);
#104987=AXIS2_PLACEMENT_3D('',#221514,#126391,#126392);
#104988=AXIS2_PLACEMENT_3D('',#221518,#126394,#126395);
#104989=AXIS2_PLACEMENT_3D('',#221520,#126396,#126397);
#104990=AXIS2_PLACEMENT_3D('',#221522,#126398,#126399);
#104991=AXIS2_PLACEMENT_3D('',#221524,#126401,#126402);
#104992=AXIS2_PLACEMENT_3D('',#221528,#126404,#126405);
#104993=AXIS2_PLACEMENT_3D('',#221530,#126407,#126408);
#104994=AXIS2_PLACEMENT_3D('',#221531,#126409,#126410);
#104995=AXIS2_PLACEMENT_3D('',#221532,#126411,#126412);
#104996=AXIS2_PLACEMENT_3D('',#221533,#126413,#126414);
#104997=AXIS2_PLACEMENT_3D('',#221534,#126415,#126416);
#104998=AXIS2_PLACEMENT_3D('',#221535,#126417,#126418);
#104999=AXIS2_PLACEMENT_3D('',#221536,#126419,#126420);
#105000=AXIS2_PLACEMENT_3D('',#221537,#126421,#126422);
#105001=AXIS2_PLACEMENT_3D('',#221538,#126423,#126424);
#105002=AXIS2_PLACEMENT_3D('',#221539,#126425,#126426);
#105003=AXIS2_PLACEMENT_3D('',#221540,#126427,#126428);
#105004=AXIS2_PLACEMENT_3D('',#221541,#126429,#126430);
#105005=AXIS2_PLACEMENT_3D('',#221542,#126431,#126432);
#105006=AXIS2_PLACEMENT_3D('',#221545,#126433,#126434);
#105007=AXIS2_PLACEMENT_3D('',#221549,#126436,#126437);
#105008=AXIS2_PLACEMENT_3D('',#221551,#126438,#126439);
#105009=AXIS2_PLACEMENT_3D('',#221553,#126440,#126441);
#105010=AXIS2_PLACEMENT_3D('',#221555,#126443,#126444);
#105011=AXIS2_PLACEMENT_3D('',#221559,#126446,#126447);
#105012=AXIS2_PLACEMENT_3D('',#221561,#126449,#126450);
#105013=AXIS2_PLACEMENT_3D('',#221564,#126451,#126452);
#105014=AXIS2_PLACEMENT_3D('',#221568,#126454,#126455);
#105015=AXIS2_PLACEMENT_3D('',#221570,#126457,#126458);
#105016=AXIS2_PLACEMENT_3D('',#221573,#126459,#126460);
#105017=AXIS2_PLACEMENT_3D('',#221577,#126462,#126463);
#105018=AXIS2_PLACEMENT_3D('',#221579,#126464,#126465);
#105019=AXIS2_PLACEMENT_3D('',#221581,#126466,#126467);
#105020=AXIS2_PLACEMENT_3D('',#221583,#126469,#126470);
#105021=AXIS2_PLACEMENT_3D('',#221587,#126472,#126473);
#105022=AXIS2_PLACEMENT_3D('',#221589,#126475,#126476);
#105023=AXIS2_PLACEMENT_3D('',#221590,#126477,#126478);
#105024=AXIS2_PLACEMENT_3D('',#221591,#126479,#126480);
#105025=AXIS2_PLACEMENT_3D('',#221592,#126481,#126482);
#105026=AXIS2_PLACEMENT_3D('',#221593,#126483,#126484);
#105027=AXIS2_PLACEMENT_3D('',#221594,#126485,#126486);
#105028=AXIS2_PLACEMENT_3D('',#221595,#126487,#126488);
#105029=AXIS2_PLACEMENT_3D('',#221596,#126489,#126490);
#105030=AXIS2_PLACEMENT_3D('',#221597,#126491,#126492);
#105031=AXIS2_PLACEMENT_3D('',#221598,#126493,#126494);
#105032=AXIS2_PLACEMENT_3D('',#221599,#126495,#126496);
#105033=AXIS2_PLACEMENT_3D('',#221600,#126497,#126498);
#105034=AXIS2_PLACEMENT_3D('',#221601,#126499,#126500);
#105035=AXIS2_PLACEMENT_3D('',#221604,#126501,#126502);
#105036=AXIS2_PLACEMENT_3D('',#221608,#126504,#126505);
#105037=AXIS2_PLACEMENT_3D('',#221610,#126506,#126507);
#105038=AXIS2_PLACEMENT_3D('',#221612,#126508,#126509);
#105039=AXIS2_PLACEMENT_3D('',#221614,#126511,#126512);
#105040=AXIS2_PLACEMENT_3D('',#221618,#126514,#126515);
#105041=AXIS2_PLACEMENT_3D('',#221620,#126517,#126518);
#105042=AXIS2_PLACEMENT_3D('',#221623,#126519,#126520);
#105043=AXIS2_PLACEMENT_3D('',#221627,#126522,#126523);
#105044=AXIS2_PLACEMENT_3D('',#221629,#126525,#126526);
#105045=AXIS2_PLACEMENT_3D('',#221632,#126527,#126528);
#105046=AXIS2_PLACEMENT_3D('',#221636,#126530,#126531);
#105047=AXIS2_PLACEMENT_3D('',#221638,#126532,#126533);
#105048=AXIS2_PLACEMENT_3D('',#221640,#126534,#126535);
#105049=AXIS2_PLACEMENT_3D('',#221642,#126537,#126538);
#105050=AXIS2_PLACEMENT_3D('',#221646,#126540,#126541);
#105051=AXIS2_PLACEMENT_3D('',#221648,#126543,#126544);
#105052=AXIS2_PLACEMENT_3D('',#221649,#126545,#126546);
#105053=AXIS2_PLACEMENT_3D('',#221650,#126547,#126548);
#105054=AXIS2_PLACEMENT_3D('',#221651,#126549,#126550);
#105055=AXIS2_PLACEMENT_3D('',#221652,#126551,#126552);
#105056=AXIS2_PLACEMENT_3D('',#221653,#126553,#126554);
#105057=AXIS2_PLACEMENT_3D('',#221654,#126555,#126556);
#105058=AXIS2_PLACEMENT_3D('',#221655,#126557,#126558);
#105059=AXIS2_PLACEMENT_3D('',#221656,#126559,#126560);
#105060=AXIS2_PLACEMENT_3D('',#221657,#126561,#126562);
#105061=AXIS2_PLACEMENT_3D('',#221658,#126563,#126564);
#105062=AXIS2_PLACEMENT_3D('',#221659,#126565,#126566);
#105063=AXIS2_PLACEMENT_3D('',#221660,#126567,#126568);
#105064=AXIS2_PLACEMENT_3D('',#221663,#126569,#126570);
#105065=AXIS2_PLACEMENT_3D('',#221667,#126572,#126573);
#105066=AXIS2_PLACEMENT_3D('',#221669,#126574,#126575);
#105067=AXIS2_PLACEMENT_3D('',#221671,#126576,#126577);
#105068=AXIS2_PLACEMENT_3D('',#221673,#126579,#126580);
#105069=AXIS2_PLACEMENT_3D('',#221677,#126582,#126583);
#105070=AXIS2_PLACEMENT_3D('',#221679,#126585,#126586);
#105071=AXIS2_PLACEMENT_3D('',#221682,#126587,#126588);
#105072=AXIS2_PLACEMENT_3D('',#221686,#126590,#126591);
#105073=AXIS2_PLACEMENT_3D('',#221688,#126593,#126594);
#105074=AXIS2_PLACEMENT_3D('',#221691,#126595,#126596);
#105075=AXIS2_PLACEMENT_3D('',#221695,#126598,#126599);
#105076=AXIS2_PLACEMENT_3D('',#221697,#126600,#126601);
#105077=AXIS2_PLACEMENT_3D('',#221699,#126602,#126603);
#105078=AXIS2_PLACEMENT_3D('',#221701,#126605,#126606);
#105079=AXIS2_PLACEMENT_3D('',#221705,#126608,#126609);
#105080=AXIS2_PLACEMENT_3D('',#221707,#126611,#126612);
#105081=AXIS2_PLACEMENT_3D('',#221708,#126613,#126614);
#105082=AXIS2_PLACEMENT_3D('',#221709,#126615,#126616);
#105083=AXIS2_PLACEMENT_3D('',#221710,#126617,#126618);
#105084=AXIS2_PLACEMENT_3D('',#221711,#126619,#126620);
#105085=AXIS2_PLACEMENT_3D('',#221712,#126621,#126622);
#105086=AXIS2_PLACEMENT_3D('',#221713,#126623,#126624);
#105087=AXIS2_PLACEMENT_3D('',#221714,#126625,#126626);
#105088=AXIS2_PLACEMENT_3D('',#221715,#126627,#126628);
#105089=AXIS2_PLACEMENT_3D('',#221716,#126629,#126630);
#105090=AXIS2_PLACEMENT_3D('',#221717,#126631,#126632);
#105091=AXIS2_PLACEMENT_3D('',#221718,#126633,#126634);
#105092=AXIS2_PLACEMENT_3D('',#221719,#126635,#126636);
#105093=AXIS2_PLACEMENT_3D('',#221722,#126637,#126638);
#105094=AXIS2_PLACEMENT_3D('',#221726,#126640,#126641);
#105095=AXIS2_PLACEMENT_3D('',#221728,#126642,#126643);
#105096=AXIS2_PLACEMENT_3D('',#221730,#126644,#126645);
#105097=AXIS2_PLACEMENT_3D('',#221732,#126647,#126648);
#105098=AXIS2_PLACEMENT_3D('',#221736,#126650,#126651);
#105099=AXIS2_PLACEMENT_3D('',#221738,#126653,#126654);
#105100=AXIS2_PLACEMENT_3D('',#221741,#126655,#126656);
#105101=AXIS2_PLACEMENT_3D('',#221745,#126658,#126659);
#105102=AXIS2_PLACEMENT_3D('',#221747,#126661,#126662);
#105103=AXIS2_PLACEMENT_3D('',#221750,#126663,#126664);
#105104=AXIS2_PLACEMENT_3D('',#221754,#126666,#126667);
#105105=AXIS2_PLACEMENT_3D('',#221756,#126668,#126669);
#105106=AXIS2_PLACEMENT_3D('',#221758,#126670,#126671);
#105107=AXIS2_PLACEMENT_3D('',#221760,#126673,#126674);
#105108=AXIS2_PLACEMENT_3D('',#221764,#126676,#126677);
#105109=AXIS2_PLACEMENT_3D('',#221766,#126679,#126680);
#105110=AXIS2_PLACEMENT_3D('',#221767,#126681,#126682);
#105111=AXIS2_PLACEMENT_3D('',#221768,#126683,#126684);
#105112=AXIS2_PLACEMENT_3D('',#221769,#126685,#126686);
#105113=AXIS2_PLACEMENT_3D('',#221770,#126687,#126688);
#105114=AXIS2_PLACEMENT_3D('',#221771,#126689,#126690);
#105115=AXIS2_PLACEMENT_3D('',#221772,#126691,#126692);
#105116=AXIS2_PLACEMENT_3D('',#221773,#126693,#126694);
#105117=AXIS2_PLACEMENT_3D('',#221774,#126695,#126696);
#105118=AXIS2_PLACEMENT_3D('',#221775,#126697,#126698);
#105119=AXIS2_PLACEMENT_3D('',#221776,#126699,#126700);
#105120=AXIS2_PLACEMENT_3D('',#221777,#126701,#126702);
#105121=AXIS2_PLACEMENT_3D('',#221778,#126703,#126704);
#105122=AXIS2_PLACEMENT_3D('',#221781,#126705,#126706);
#105123=AXIS2_PLACEMENT_3D('',#221785,#126708,#126709);
#105124=AXIS2_PLACEMENT_3D('',#221787,#126710,#126711);
#105125=AXIS2_PLACEMENT_3D('',#221789,#126712,#126713);
#105126=AXIS2_PLACEMENT_3D('',#221791,#126715,#126716);
#105127=AXIS2_PLACEMENT_3D('',#221795,#126718,#126719);
#105128=AXIS2_PLACEMENT_3D('',#221797,#126721,#126722);
#105129=AXIS2_PLACEMENT_3D('',#221800,#126723,#126724);
#105130=AXIS2_PLACEMENT_3D('',#221804,#126726,#126727);
#105131=AXIS2_PLACEMENT_3D('',#221806,#126729,#126730);
#105132=AXIS2_PLACEMENT_3D('',#221809,#126731,#126732);
#105133=AXIS2_PLACEMENT_3D('',#221813,#126734,#126735);
#105134=AXIS2_PLACEMENT_3D('',#221815,#126736,#126737);
#105135=AXIS2_PLACEMENT_3D('',#221817,#126738,#126739);
#105136=AXIS2_PLACEMENT_3D('',#221819,#126741,#126742);
#105137=AXIS2_PLACEMENT_3D('',#221823,#126744,#126745);
#105138=AXIS2_PLACEMENT_3D('',#221825,#126747,#126748);
#105139=AXIS2_PLACEMENT_3D('',#221826,#126749,#126750);
#105140=AXIS2_PLACEMENT_3D('',#221827,#126751,#126752);
#105141=AXIS2_PLACEMENT_3D('',#221828,#126753,#126754);
#105142=AXIS2_PLACEMENT_3D('',#221829,#126755,#126756);
#105143=AXIS2_PLACEMENT_3D('',#221830,#126757,#126758);
#105144=AXIS2_PLACEMENT_3D('',#221831,#126759,#126760);
#105145=AXIS2_PLACEMENT_3D('',#221832,#126761,#126762);
#105146=AXIS2_PLACEMENT_3D('',#221833,#126763,#126764);
#105147=AXIS2_PLACEMENT_3D('',#221834,#126765,#126766);
#105148=AXIS2_PLACEMENT_3D('',#221835,#126767,#126768);
#105149=AXIS2_PLACEMENT_3D('',#221836,#126769,#126770);
#105150=AXIS2_PLACEMENT_3D('',#221837,#126771,#126772);
#105151=AXIS2_PLACEMENT_3D('',#221840,#126773,#126774);
#105152=AXIS2_PLACEMENT_3D('',#221844,#126776,#126777);
#105153=AXIS2_PLACEMENT_3D('',#221846,#126778,#126779);
#105154=AXIS2_PLACEMENT_3D('',#221848,#126780,#126781);
#105155=AXIS2_PLACEMENT_3D('',#221850,#126783,#126784);
#105156=AXIS2_PLACEMENT_3D('',#221854,#126786,#126787);
#105157=AXIS2_PLACEMENT_3D('',#221856,#126789,#126790);
#105158=AXIS2_PLACEMENT_3D('',#221859,#126791,#126792);
#105159=AXIS2_PLACEMENT_3D('',#221863,#126794,#126795);
#105160=AXIS2_PLACEMENT_3D('',#221865,#126797,#126798);
#105161=AXIS2_PLACEMENT_3D('',#221868,#126799,#126800);
#105162=AXIS2_PLACEMENT_3D('',#221872,#126802,#126803);
#105163=AXIS2_PLACEMENT_3D('',#221874,#126804,#126805);
#105164=AXIS2_PLACEMENT_3D('',#221876,#126806,#126807);
#105165=AXIS2_PLACEMENT_3D('',#221878,#126809,#126810);
#105166=AXIS2_PLACEMENT_3D('',#221882,#126812,#126813);
#105167=AXIS2_PLACEMENT_3D('',#221884,#126815,#126816);
#105168=AXIS2_PLACEMENT_3D('',#221885,#126817,#126818);
#105169=AXIS2_PLACEMENT_3D('',#221886,#126819,#126820);
#105170=AXIS2_PLACEMENT_3D('',#221887,#126821,#126822);
#105171=AXIS2_PLACEMENT_3D('',#221888,#126823,#126824);
#105172=AXIS2_PLACEMENT_3D('',#221889,#126825,#126826);
#105173=AXIS2_PLACEMENT_3D('',#221890,#126827,#126828);
#105174=AXIS2_PLACEMENT_3D('',#221891,#126829,#126830);
#105175=AXIS2_PLACEMENT_3D('',#221892,#126831,#126832);
#105176=AXIS2_PLACEMENT_3D('',#221893,#126833,#126834);
#105177=AXIS2_PLACEMENT_3D('',#221894,#126835,#126836);
#105178=AXIS2_PLACEMENT_3D('',#221895,#126837,#126838);
#105179=AXIS2_PLACEMENT_3D('',#221896,#126839,#126840);
#105180=AXIS2_PLACEMENT_3D('',#221899,#126841,#126842);
#105181=AXIS2_PLACEMENT_3D('',#221903,#126844,#126845);
#105182=AXIS2_PLACEMENT_3D('',#221905,#126846,#126847);
#105183=AXIS2_PLACEMENT_3D('',#221907,#126848,#126849);
#105184=AXIS2_PLACEMENT_3D('',#221909,#126851,#126852);
#105185=AXIS2_PLACEMENT_3D('',#221913,#126854,#126855);
#105186=AXIS2_PLACEMENT_3D('',#221915,#126857,#126858);
#105187=AXIS2_PLACEMENT_3D('',#221918,#126859,#126860);
#105188=AXIS2_PLACEMENT_3D('',#221922,#126862,#126863);
#105189=AXIS2_PLACEMENT_3D('',#221924,#126865,#126866);
#105190=AXIS2_PLACEMENT_3D('',#221927,#126867,#126868);
#105191=AXIS2_PLACEMENT_3D('',#221931,#126870,#126871);
#105192=AXIS2_PLACEMENT_3D('',#221933,#126872,#126873);
#105193=AXIS2_PLACEMENT_3D('',#221935,#126874,#126875);
#105194=AXIS2_PLACEMENT_3D('',#221937,#126877,#126878);
#105195=AXIS2_PLACEMENT_3D('',#221941,#126880,#126881);
#105196=AXIS2_PLACEMENT_3D('',#221943,#126883,#126884);
#105197=AXIS2_PLACEMENT_3D('',#221944,#126885,#126886);
#105198=AXIS2_PLACEMENT_3D('',#221945,#126887,#126888);
#105199=AXIS2_PLACEMENT_3D('',#221946,#126889,#126890);
#105200=AXIS2_PLACEMENT_3D('',#221947,#126891,#126892);
#105201=AXIS2_PLACEMENT_3D('',#221948,#126893,#126894);
#105202=AXIS2_PLACEMENT_3D('',#221949,#126895,#126896);
#105203=AXIS2_PLACEMENT_3D('',#221950,#126897,#126898);
#105204=AXIS2_PLACEMENT_3D('',#221951,#126899,#126900);
#105205=AXIS2_PLACEMENT_3D('',#221952,#126901,#126902);
#105206=AXIS2_PLACEMENT_3D('',#221953,#126903,#126904);
#105207=AXIS2_PLACEMENT_3D('',#221954,#126905,#126906);
#105208=AXIS2_PLACEMENT_3D('',#221955,#126907,#126908);
#105209=AXIS2_PLACEMENT_3D('',#221958,#126909,#126910);
#105210=AXIS2_PLACEMENT_3D('',#221962,#126912,#126913);
#105211=AXIS2_PLACEMENT_3D('',#221964,#126914,#126915);
#105212=AXIS2_PLACEMENT_3D('',#221966,#126916,#126917);
#105213=AXIS2_PLACEMENT_3D('',#221968,#126919,#126920);
#105214=AXIS2_PLACEMENT_3D('',#221972,#126922,#126923);
#105215=AXIS2_PLACEMENT_3D('',#221974,#126925,#126926);
#105216=AXIS2_PLACEMENT_3D('',#221977,#126927,#126928);
#105217=AXIS2_PLACEMENT_3D('',#221981,#126930,#126931);
#105218=AXIS2_PLACEMENT_3D('',#221983,#126933,#126934);
#105219=AXIS2_PLACEMENT_3D('',#221986,#126935,#126936);
#105220=AXIS2_PLACEMENT_3D('',#221990,#126938,#126939);
#105221=AXIS2_PLACEMENT_3D('',#221992,#126940,#126941);
#105222=AXIS2_PLACEMENT_3D('',#221994,#126942,#126943);
#105223=AXIS2_PLACEMENT_3D('',#221996,#126945,#126946);
#105224=AXIS2_PLACEMENT_3D('',#222000,#126948,#126949);
#105225=AXIS2_PLACEMENT_3D('',#222002,#126951,#126952);
#105226=AXIS2_PLACEMENT_3D('',#222003,#126953,#126954);
#105227=AXIS2_PLACEMENT_3D('',#222004,#126955,#126956);
#105228=AXIS2_PLACEMENT_3D('',#222005,#126957,#126958);
#105229=AXIS2_PLACEMENT_3D('',#222006,#126959,#126960);
#105230=AXIS2_PLACEMENT_3D('',#222007,#126961,#126962);
#105231=AXIS2_PLACEMENT_3D('',#222008,#126963,#126964);
#105232=AXIS2_PLACEMENT_3D('',#222009,#126965,#126966);
#105233=AXIS2_PLACEMENT_3D('',#222010,#126967,#126968);
#105234=AXIS2_PLACEMENT_3D('',#222011,#126969,#126970);
#105235=AXIS2_PLACEMENT_3D('',#222012,#126971,#126972);
#105236=AXIS2_PLACEMENT_3D('',#222013,#126973,#126974);
#105237=AXIS2_PLACEMENT_3D('',#222014,#126975,#126976);
#105238=AXIS2_PLACEMENT_3D('',#222017,#126977,#126978);
#105239=AXIS2_PLACEMENT_3D('',#222021,#126980,#126981);
#105240=AXIS2_PLACEMENT_3D('',#222023,#126982,#126983);
#105241=AXIS2_PLACEMENT_3D('',#222025,#126984,#126985);
#105242=AXIS2_PLACEMENT_3D('',#222027,#126987,#126988);
#105243=AXIS2_PLACEMENT_3D('',#222031,#126990,#126991);
#105244=AXIS2_PLACEMENT_3D('',#222033,#126993,#126994);
#105245=AXIS2_PLACEMENT_3D('',#222036,#126995,#126996);
#105246=AXIS2_PLACEMENT_3D('',#222040,#126998,#126999);
#105247=AXIS2_PLACEMENT_3D('',#222042,#127001,#127002);
#105248=AXIS2_PLACEMENT_3D('',#222045,#127003,#127004);
#105249=AXIS2_PLACEMENT_3D('',#222049,#127006,#127007);
#105250=AXIS2_PLACEMENT_3D('',#222051,#127008,#127009);
#105251=AXIS2_PLACEMENT_3D('',#222053,#127010,#127011);
#105252=AXIS2_PLACEMENT_3D('',#222055,#127013,#127014);
#105253=AXIS2_PLACEMENT_3D('',#222059,#127016,#127017);
#105254=AXIS2_PLACEMENT_3D('',#222061,#127019,#127020);
#105255=AXIS2_PLACEMENT_3D('',#222062,#127021,#127022);
#105256=AXIS2_PLACEMENT_3D('',#222063,#127023,#127024);
#105257=AXIS2_PLACEMENT_3D('',#222064,#127025,#127026);
#105258=AXIS2_PLACEMENT_3D('',#222065,#127027,#127028);
#105259=AXIS2_PLACEMENT_3D('',#222066,#127029,#127030);
#105260=AXIS2_PLACEMENT_3D('',#222067,#127031,#127032);
#105261=AXIS2_PLACEMENT_3D('',#222068,#127033,#127034);
#105262=AXIS2_PLACEMENT_3D('',#222069,#127035,#127036);
#105263=AXIS2_PLACEMENT_3D('',#222070,#127037,#127038);
#105264=AXIS2_PLACEMENT_3D('',#222071,#127039,#127040);
#105265=AXIS2_PLACEMENT_3D('',#222072,#127041,#127042);
#105266=AXIS2_PLACEMENT_3D('',#222073,#127043,#127044);
#105267=AXIS2_PLACEMENT_3D('',#222076,#127045,#127046);
#105268=AXIS2_PLACEMENT_3D('',#222080,#127048,#127049);
#105269=AXIS2_PLACEMENT_3D('',#222082,#127050,#127051);
#105270=AXIS2_PLACEMENT_3D('',#222084,#127052,#127053);
#105271=AXIS2_PLACEMENT_3D('',#222086,#127055,#127056);
#105272=AXIS2_PLACEMENT_3D('',#222090,#127058,#127059);
#105273=AXIS2_PLACEMENT_3D('',#222092,#127061,#127062);
#105274=AXIS2_PLACEMENT_3D('',#222095,#127063,#127064);
#105275=AXIS2_PLACEMENT_3D('',#222099,#127066,#127067);
#105276=AXIS2_PLACEMENT_3D('',#222101,#127069,#127070);
#105277=AXIS2_PLACEMENT_3D('',#222104,#127071,#127072);
#105278=AXIS2_PLACEMENT_3D('',#222108,#127074,#127075);
#105279=AXIS2_PLACEMENT_3D('',#222110,#127076,#127077);
#105280=AXIS2_PLACEMENT_3D('',#222112,#127078,#127079);
#105281=AXIS2_PLACEMENT_3D('',#222114,#127081,#127082);
#105282=AXIS2_PLACEMENT_3D('',#222118,#127084,#127085);
#105283=AXIS2_PLACEMENT_3D('',#222120,#127087,#127088);
#105284=AXIS2_PLACEMENT_3D('',#222121,#127089,#127090);
#105285=AXIS2_PLACEMENT_3D('',#222122,#127091,#127092);
#105286=AXIS2_PLACEMENT_3D('',#222123,#127093,#127094);
#105287=AXIS2_PLACEMENT_3D('',#222124,#127095,#127096);
#105288=AXIS2_PLACEMENT_3D('',#222125,#127097,#127098);
#105289=AXIS2_PLACEMENT_3D('',#222126,#127099,#127100);
#105290=AXIS2_PLACEMENT_3D('',#222127,#127101,#127102);
#105291=AXIS2_PLACEMENT_3D('',#222128,#127103,#127104);
#105292=AXIS2_PLACEMENT_3D('',#222129,#127105,#127106);
#105293=AXIS2_PLACEMENT_3D('',#222130,#127107,#127108);
#105294=AXIS2_PLACEMENT_3D('',#222131,#127109,#127110);
#105295=AXIS2_PLACEMENT_3D('',#222132,#127111,#127112);
#105296=AXIS2_PLACEMENT_3D('',#222135,#127113,#127114);
#105297=AXIS2_PLACEMENT_3D('',#222139,#127116,#127117);
#105298=AXIS2_PLACEMENT_3D('',#222141,#127118,#127119);
#105299=AXIS2_PLACEMENT_3D('',#222143,#127120,#127121);
#105300=AXIS2_PLACEMENT_3D('',#222145,#127123,#127124);
#105301=AXIS2_PLACEMENT_3D('',#222149,#127126,#127127);
#105302=AXIS2_PLACEMENT_3D('',#222151,#127129,#127130);
#105303=AXIS2_PLACEMENT_3D('',#222154,#127131,#127132);
#105304=AXIS2_PLACEMENT_3D('',#222158,#127134,#127135);
#105305=AXIS2_PLACEMENT_3D('',#222160,#127137,#127138);
#105306=AXIS2_PLACEMENT_3D('',#222163,#127139,#127140);
#105307=AXIS2_PLACEMENT_3D('',#222167,#127142,#127143);
#105308=AXIS2_PLACEMENT_3D('',#222169,#127144,#127145);
#105309=AXIS2_PLACEMENT_3D('',#222171,#127146,#127147);
#105310=AXIS2_PLACEMENT_3D('',#222173,#127149,#127150);
#105311=AXIS2_PLACEMENT_3D('',#222177,#127152,#127153);
#105312=AXIS2_PLACEMENT_3D('',#222179,#127155,#127156);
#105313=AXIS2_PLACEMENT_3D('',#222180,#127157,#127158);
#105314=AXIS2_PLACEMENT_3D('',#222181,#127159,#127160);
#105315=AXIS2_PLACEMENT_3D('',#222182,#127161,#127162);
#105316=AXIS2_PLACEMENT_3D('',#222183,#127163,#127164);
#105317=AXIS2_PLACEMENT_3D('',#222184,#127165,#127166);
#105318=AXIS2_PLACEMENT_3D('',#222185,#127167,#127168);
#105319=AXIS2_PLACEMENT_3D('',#222186,#127169,#127170);
#105320=AXIS2_PLACEMENT_3D('',#222187,#127171,#127172);
#105321=AXIS2_PLACEMENT_3D('',#222188,#127173,#127174);
#105322=AXIS2_PLACEMENT_3D('',#222189,#127175,#127176);
#105323=AXIS2_PLACEMENT_3D('',#222190,#127177,#127178);
#105324=AXIS2_PLACEMENT_3D('',#222191,#127179,#127180);
#105325=AXIS2_PLACEMENT_3D('',#222194,#127181,#127182);
#105326=AXIS2_PLACEMENT_3D('',#222198,#127184,#127185);
#105327=AXIS2_PLACEMENT_3D('',#222200,#127186,#127187);
#105328=AXIS2_PLACEMENT_3D('',#222202,#127188,#127189);
#105329=AXIS2_PLACEMENT_3D('',#222204,#127191,#127192);
#105330=AXIS2_PLACEMENT_3D('',#222208,#127194,#127195);
#105331=AXIS2_PLACEMENT_3D('',#222210,#127197,#127198);
#105332=AXIS2_PLACEMENT_3D('',#222213,#127199,#127200);
#105333=AXIS2_PLACEMENT_3D('',#222217,#127202,#127203);
#105334=AXIS2_PLACEMENT_3D('',#222219,#127205,#127206);
#105335=AXIS2_PLACEMENT_3D('',#222222,#127207,#127208);
#105336=AXIS2_PLACEMENT_3D('',#222226,#127210,#127211);
#105337=AXIS2_PLACEMENT_3D('',#222228,#127212,#127213);
#105338=AXIS2_PLACEMENT_3D('',#222230,#127214,#127215);
#105339=AXIS2_PLACEMENT_3D('',#222232,#127217,#127218);
#105340=AXIS2_PLACEMENT_3D('',#222236,#127220,#127221);
#105341=AXIS2_PLACEMENT_3D('',#222238,#127223,#127224);
#105342=AXIS2_PLACEMENT_3D('',#222239,#127225,#127226);
#105343=AXIS2_PLACEMENT_3D('',#222240,#127227,#127228);
#105344=AXIS2_PLACEMENT_3D('',#222241,#127229,#127230);
#105345=AXIS2_PLACEMENT_3D('',#222242,#127231,#127232);
#105346=AXIS2_PLACEMENT_3D('',#222243,#127233,#127234);
#105347=AXIS2_PLACEMENT_3D('',#222244,#127235,#127236);
#105348=AXIS2_PLACEMENT_3D('',#222245,#127237,#127238);
#105349=AXIS2_PLACEMENT_3D('',#222246,#127239,#127240);
#105350=AXIS2_PLACEMENT_3D('',#222247,#127241,#127242);
#105351=AXIS2_PLACEMENT_3D('',#222248,#127243,#127244);
#105352=AXIS2_PLACEMENT_3D('',#222249,#127245,#127246);
#105353=AXIS2_PLACEMENT_3D('',#222250,#127247,#127248);
#105354=AXIS2_PLACEMENT_3D('',#222253,#127249,#127250);
#105355=AXIS2_PLACEMENT_3D('',#222257,#127252,#127253);
#105356=AXIS2_PLACEMENT_3D('',#222259,#127254,#127255);
#105357=AXIS2_PLACEMENT_3D('',#222261,#127256,#127257);
#105358=AXIS2_PLACEMENT_3D('',#222263,#127259,#127260);
#105359=AXIS2_PLACEMENT_3D('',#222267,#127262,#127263);
#105360=AXIS2_PLACEMENT_3D('',#222269,#127265,#127266);
#105361=AXIS2_PLACEMENT_3D('',#222272,#127267,#127268);
#105362=AXIS2_PLACEMENT_3D('',#222276,#127270,#127271);
#105363=AXIS2_PLACEMENT_3D('',#222278,#127273,#127274);
#105364=AXIS2_PLACEMENT_3D('',#222281,#127275,#127276);
#105365=AXIS2_PLACEMENT_3D('',#222285,#127278,#127279);
#105366=AXIS2_PLACEMENT_3D('',#222287,#127280,#127281);
#105367=AXIS2_PLACEMENT_3D('',#222289,#127282,#127283);
#105368=AXIS2_PLACEMENT_3D('',#222291,#127285,#127286);
#105369=AXIS2_PLACEMENT_3D('',#222295,#127288,#127289);
#105370=AXIS2_PLACEMENT_3D('',#222297,#127291,#127292);
#105371=AXIS2_PLACEMENT_3D('',#222298,#127293,#127294);
#105372=AXIS2_PLACEMENT_3D('',#222299,#127295,#127296);
#105373=AXIS2_PLACEMENT_3D('',#222300,#127297,#127298);
#105374=AXIS2_PLACEMENT_3D('',#222301,#127299,#127300);
#105375=AXIS2_PLACEMENT_3D('',#222302,#127301,#127302);
#105376=AXIS2_PLACEMENT_3D('',#222303,#127303,#127304);
#105377=AXIS2_PLACEMENT_3D('',#222304,#127305,#127306);
#105378=AXIS2_PLACEMENT_3D('',#222305,#127307,#127308);
#105379=AXIS2_PLACEMENT_3D('',#222306,#127309,#127310);
#105380=AXIS2_PLACEMENT_3D('',#222307,#127311,#127312);
#105381=AXIS2_PLACEMENT_3D('',#222308,#127313,#127314);
#105382=AXIS2_PLACEMENT_3D('',#222309,#127315,#127316);
#105383=AXIS2_PLACEMENT_3D('',#222312,#127317,#127318);
#105384=AXIS2_PLACEMENT_3D('',#222316,#127320,#127321);
#105385=AXIS2_PLACEMENT_3D('',#222318,#127322,#127323);
#105386=AXIS2_PLACEMENT_3D('',#222320,#127324,#127325);
#105387=AXIS2_PLACEMENT_3D('',#222322,#127327,#127328);
#105388=AXIS2_PLACEMENT_3D('',#222326,#127330,#127331);
#105389=AXIS2_PLACEMENT_3D('',#222328,#127333,#127334);
#105390=AXIS2_PLACEMENT_3D('',#222331,#127335,#127336);
#105391=AXIS2_PLACEMENT_3D('',#222335,#127338,#127339);
#105392=AXIS2_PLACEMENT_3D('',#222337,#127341,#127342);
#105393=AXIS2_PLACEMENT_3D('',#222340,#127343,#127344);
#105394=AXIS2_PLACEMENT_3D('',#222344,#127346,#127347);
#105395=AXIS2_PLACEMENT_3D('',#222346,#127348,#127349);
#105396=AXIS2_PLACEMENT_3D('',#222348,#127350,#127351);
#105397=AXIS2_PLACEMENT_3D('',#222350,#127353,#127354);
#105398=AXIS2_PLACEMENT_3D('',#222354,#127356,#127357);
#105399=AXIS2_PLACEMENT_3D('',#222356,#127359,#127360);
#105400=AXIS2_PLACEMENT_3D('',#222357,#127361,#127362);
#105401=AXIS2_PLACEMENT_3D('',#222358,#127363,#127364);
#105402=AXIS2_PLACEMENT_3D('',#222359,#127365,#127366);
#105403=AXIS2_PLACEMENT_3D('',#222360,#127367,#127368);
#105404=AXIS2_PLACEMENT_3D('',#222361,#127369,#127370);
#105405=AXIS2_PLACEMENT_3D('',#222362,#127371,#127372);
#105406=AXIS2_PLACEMENT_3D('',#222363,#127373,#127374);
#105407=AXIS2_PLACEMENT_3D('',#222364,#127375,#127376);
#105408=AXIS2_PLACEMENT_3D('',#222365,#127377,#127378);
#105409=AXIS2_PLACEMENT_3D('',#222366,#127379,#127380);
#105410=AXIS2_PLACEMENT_3D('',#222367,#127381,#127382);
#105411=AXIS2_PLACEMENT_3D('',#222368,#127383,#127384);
#105412=AXIS2_PLACEMENT_3D('',#222371,#127385,#127386);
#105413=AXIS2_PLACEMENT_3D('',#222375,#127388,#127389);
#105414=AXIS2_PLACEMENT_3D('',#222377,#127390,#127391);
#105415=AXIS2_PLACEMENT_3D('',#222379,#127392,#127393);
#105416=AXIS2_PLACEMENT_3D('',#222381,#127395,#127396);
#105417=AXIS2_PLACEMENT_3D('',#222385,#127398,#127399);
#105418=AXIS2_PLACEMENT_3D('',#222387,#127401,#127402);
#105419=AXIS2_PLACEMENT_3D('',#222390,#127403,#127404);
#105420=AXIS2_PLACEMENT_3D('',#222394,#127406,#127407);
#105421=AXIS2_PLACEMENT_3D('',#222396,#127409,#127410);
#105422=AXIS2_PLACEMENT_3D('',#222399,#127411,#127412);
#105423=AXIS2_PLACEMENT_3D('',#222403,#127414,#127415);
#105424=AXIS2_PLACEMENT_3D('',#222405,#127416,#127417);
#105425=AXIS2_PLACEMENT_3D('',#222407,#127418,#127419);
#105426=AXIS2_PLACEMENT_3D('',#222409,#127421,#127422);
#105427=AXIS2_PLACEMENT_3D('',#222413,#127424,#127425);
#105428=AXIS2_PLACEMENT_3D('',#222415,#127427,#127428);
#105429=AXIS2_PLACEMENT_3D('',#222416,#127429,#127430);
#105430=AXIS2_PLACEMENT_3D('',#222417,#127431,#127432);
#105431=AXIS2_PLACEMENT_3D('',#222418,#127433,#127434);
#105432=AXIS2_PLACEMENT_3D('',#222419,#127435,#127436);
#105433=AXIS2_PLACEMENT_3D('',#222420,#127437,#127438);
#105434=AXIS2_PLACEMENT_3D('',#222421,#127439,#127440);
#105435=AXIS2_PLACEMENT_3D('',#222422,#127441,#127442);
#105436=AXIS2_PLACEMENT_3D('',#222423,#127443,#127444);
#105437=AXIS2_PLACEMENT_3D('',#222424,#127445,#127446);
#105438=AXIS2_PLACEMENT_3D('',#222425,#127447,#127448);
#105439=AXIS2_PLACEMENT_3D('',#222426,#127449,#127450);
#105440=AXIS2_PLACEMENT_3D('',#222427,#127451,#127452);
#105441=AXIS2_PLACEMENT_3D('',#222430,#127453,#127454);
#105442=AXIS2_PLACEMENT_3D('',#222434,#127456,#127457);
#105443=AXIS2_PLACEMENT_3D('',#222436,#127458,#127459);
#105444=AXIS2_PLACEMENT_3D('',#222438,#127460,#127461);
#105445=AXIS2_PLACEMENT_3D('',#222440,#127463,#127464);
#105446=AXIS2_PLACEMENT_3D('',#222444,#127466,#127467);
#105447=AXIS2_PLACEMENT_3D('',#222446,#127469,#127470);
#105448=AXIS2_PLACEMENT_3D('',#222449,#127471,#127472);
#105449=AXIS2_PLACEMENT_3D('',#222453,#127474,#127475);
#105450=AXIS2_PLACEMENT_3D('',#222455,#127477,#127478);
#105451=AXIS2_PLACEMENT_3D('',#222458,#127479,#127480);
#105452=AXIS2_PLACEMENT_3D('',#222462,#127482,#127483);
#105453=AXIS2_PLACEMENT_3D('',#222464,#127484,#127485);
#105454=AXIS2_PLACEMENT_3D('',#222466,#127486,#127487);
#105455=AXIS2_PLACEMENT_3D('',#222468,#127489,#127490);
#105456=AXIS2_PLACEMENT_3D('',#222472,#127492,#127493);
#105457=AXIS2_PLACEMENT_3D('',#222474,#127495,#127496);
#105458=AXIS2_PLACEMENT_3D('',#222475,#127497,#127498);
#105459=AXIS2_PLACEMENT_3D('',#222476,#127499,#127500);
#105460=AXIS2_PLACEMENT_3D('',#222477,#127501,#127502);
#105461=AXIS2_PLACEMENT_3D('',#222478,#127503,#127504);
#105462=AXIS2_PLACEMENT_3D('',#222479,#127505,#127506);
#105463=AXIS2_PLACEMENT_3D('',#222480,#127507,#127508);
#105464=AXIS2_PLACEMENT_3D('',#222481,#127509,#127510);
#105465=AXIS2_PLACEMENT_3D('',#222482,#127511,#127512);
#105466=AXIS2_PLACEMENT_3D('',#222483,#127513,#127514);
#105467=AXIS2_PLACEMENT_3D('',#222484,#127515,#127516);
#105468=AXIS2_PLACEMENT_3D('',#222485,#127517,#127518);
#105469=AXIS2_PLACEMENT_3D('',#222486,#127519,#127520);
#105470=AXIS2_PLACEMENT_3D('',#222489,#127521,#127522);
#105471=AXIS2_PLACEMENT_3D('',#222493,#127524,#127525);
#105472=AXIS2_PLACEMENT_3D('',#222495,#127526,#127527);
#105473=AXIS2_PLACEMENT_3D('',#222497,#127528,#127529);
#105474=AXIS2_PLACEMENT_3D('',#222499,#127531,#127532);
#105475=AXIS2_PLACEMENT_3D('',#222503,#127534,#127535);
#105476=AXIS2_PLACEMENT_3D('',#222505,#127537,#127538);
#105477=AXIS2_PLACEMENT_3D('',#222508,#127539,#127540);
#105478=AXIS2_PLACEMENT_3D('',#222512,#127542,#127543);
#105479=AXIS2_PLACEMENT_3D('',#222514,#127545,#127546);
#105480=AXIS2_PLACEMENT_3D('',#222517,#127547,#127548);
#105481=AXIS2_PLACEMENT_3D('',#222521,#127550,#127551);
#105482=AXIS2_PLACEMENT_3D('',#222523,#127552,#127553);
#105483=AXIS2_PLACEMENT_3D('',#222525,#127554,#127555);
#105484=AXIS2_PLACEMENT_3D('',#222527,#127557,#127558);
#105485=AXIS2_PLACEMENT_3D('',#222531,#127560,#127561);
#105486=AXIS2_PLACEMENT_3D('',#222533,#127563,#127564);
#105487=AXIS2_PLACEMENT_3D('',#222534,#127565,#127566);
#105488=AXIS2_PLACEMENT_3D('',#222535,#127567,#127568);
#105489=AXIS2_PLACEMENT_3D('',#222536,#127569,#127570);
#105490=AXIS2_PLACEMENT_3D('',#222537,#127571,#127572);
#105491=AXIS2_PLACEMENT_3D('',#222538,#127573,#127574);
#105492=AXIS2_PLACEMENT_3D('',#222539,#127575,#127576);
#105493=AXIS2_PLACEMENT_3D('',#222540,#127577,#127578);
#105494=AXIS2_PLACEMENT_3D('',#222541,#127579,#127580);
#105495=AXIS2_PLACEMENT_3D('',#222542,#127581,#127582);
#105496=AXIS2_PLACEMENT_3D('',#222543,#127583,#127584);
#105497=AXIS2_PLACEMENT_3D('',#222544,#127585,#127586);
#105498=AXIS2_PLACEMENT_3D('',#222545,#127587,#127588);
#105499=AXIS2_PLACEMENT_3D('',#222548,#127589,#127590);
#105500=AXIS2_PLACEMENT_3D('',#222552,#127592,#127593);
#105501=AXIS2_PLACEMENT_3D('',#222554,#127594,#127595);
#105502=AXIS2_PLACEMENT_3D('',#222556,#127596,#127597);
#105503=AXIS2_PLACEMENT_3D('',#222558,#127599,#127600);
#105504=AXIS2_PLACEMENT_3D('',#222562,#127602,#127603);
#105505=AXIS2_PLACEMENT_3D('',#222564,#127605,#127606);
#105506=AXIS2_PLACEMENT_3D('',#222567,#127607,#127608);
#105507=AXIS2_PLACEMENT_3D('',#222571,#127610,#127611);
#105508=AXIS2_PLACEMENT_3D('',#222573,#127613,#127614);
#105509=AXIS2_PLACEMENT_3D('',#222576,#127615,#127616);
#105510=AXIS2_PLACEMENT_3D('',#222580,#127618,#127619);
#105511=AXIS2_PLACEMENT_3D('',#222582,#127620,#127621);
#105512=AXIS2_PLACEMENT_3D('',#222584,#127622,#127623);
#105513=AXIS2_PLACEMENT_3D('',#222586,#127625,#127626);
#105514=AXIS2_PLACEMENT_3D('',#222590,#127628,#127629);
#105515=AXIS2_PLACEMENT_3D('',#222592,#127631,#127632);
#105516=AXIS2_PLACEMENT_3D('',#222593,#127633,#127634);
#105517=AXIS2_PLACEMENT_3D('',#222594,#127635,#127636);
#105518=AXIS2_PLACEMENT_3D('',#222595,#127637,#127638);
#105519=AXIS2_PLACEMENT_3D('',#222596,#127639,#127640);
#105520=AXIS2_PLACEMENT_3D('',#222597,#127641,#127642);
#105521=AXIS2_PLACEMENT_3D('',#222598,#127643,#127644);
#105522=AXIS2_PLACEMENT_3D('',#222599,#127645,#127646);
#105523=AXIS2_PLACEMENT_3D('',#222600,#127647,#127648);
#105524=AXIS2_PLACEMENT_3D('',#222601,#127649,#127650);
#105525=AXIS2_PLACEMENT_3D('',#222602,#127651,#127652);
#105526=AXIS2_PLACEMENT_3D('',#222603,#127653,#127654);
#105527=AXIS2_PLACEMENT_3D('',#222604,#127655,#127656);
#105528=AXIS2_PLACEMENT_3D('',#222607,#127657,#127658);
#105529=AXIS2_PLACEMENT_3D('',#222611,#127660,#127661);
#105530=AXIS2_PLACEMENT_3D('',#222613,#127662,#127663);
#105531=AXIS2_PLACEMENT_3D('',#222615,#127664,#127665);
#105532=AXIS2_PLACEMENT_3D('',#222617,#127667,#127668);
#105533=AXIS2_PLACEMENT_3D('',#222621,#127670,#127671);
#105534=AXIS2_PLACEMENT_3D('',#222623,#127673,#127674);
#105535=AXIS2_PLACEMENT_3D('',#222626,#127675,#127676);
#105536=AXIS2_PLACEMENT_3D('',#222630,#127678,#127679);
#105537=AXIS2_PLACEMENT_3D('',#222632,#127681,#127682);
#105538=AXIS2_PLACEMENT_3D('',#222635,#127683,#127684);
#105539=AXIS2_PLACEMENT_3D('',#222639,#127686,#127687);
#105540=AXIS2_PLACEMENT_3D('',#222641,#127688,#127689);
#105541=AXIS2_PLACEMENT_3D('',#222643,#127690,#127691);
#105542=AXIS2_PLACEMENT_3D('',#222645,#127693,#127694);
#105543=AXIS2_PLACEMENT_3D('',#222649,#127696,#127697);
#105544=AXIS2_PLACEMENT_3D('',#222651,#127699,#127700);
#105545=AXIS2_PLACEMENT_3D('',#222652,#127701,#127702);
#105546=AXIS2_PLACEMENT_3D('',#222653,#127703,#127704);
#105547=AXIS2_PLACEMENT_3D('',#222654,#127705,#127706);
#105548=AXIS2_PLACEMENT_3D('',#222655,#127707,#127708);
#105549=AXIS2_PLACEMENT_3D('',#222656,#127709,#127710);
#105550=AXIS2_PLACEMENT_3D('',#222657,#127711,#127712);
#105551=AXIS2_PLACEMENT_3D('',#222658,#127713,#127714);
#105552=AXIS2_PLACEMENT_3D('',#222659,#127715,#127716);
#105553=AXIS2_PLACEMENT_3D('',#222660,#127717,#127718);
#105554=AXIS2_PLACEMENT_3D('',#222661,#127719,#127720);
#105555=AXIS2_PLACEMENT_3D('',#222662,#127721,#127722);
#105556=AXIS2_PLACEMENT_3D('',#222663,#127723,#127724);
#105557=AXIS2_PLACEMENT_3D('',#222666,#127725,#127726);
#105558=AXIS2_PLACEMENT_3D('',#222670,#127728,#127729);
#105559=AXIS2_PLACEMENT_3D('',#222672,#127730,#127731);
#105560=AXIS2_PLACEMENT_3D('',#222674,#127732,#127733);
#105561=AXIS2_PLACEMENT_3D('',#222676,#127735,#127736);
#105562=AXIS2_PLACEMENT_3D('',#222680,#127738,#127739);
#105563=AXIS2_PLACEMENT_3D('',#222682,#127741,#127742);
#105564=AXIS2_PLACEMENT_3D('',#222685,#127743,#127744);
#105565=AXIS2_PLACEMENT_3D('',#222689,#127746,#127747);
#105566=AXIS2_PLACEMENT_3D('',#222691,#127749,#127750);
#105567=AXIS2_PLACEMENT_3D('',#222694,#127751,#127752);
#105568=AXIS2_PLACEMENT_3D('',#222698,#127754,#127755);
#105569=AXIS2_PLACEMENT_3D('',#222700,#127756,#127757);
#105570=AXIS2_PLACEMENT_3D('',#222702,#127758,#127759);
#105571=AXIS2_PLACEMENT_3D('',#222704,#127761,#127762);
#105572=AXIS2_PLACEMENT_3D('',#222708,#127764,#127765);
#105573=AXIS2_PLACEMENT_3D('',#222710,#127767,#127768);
#105574=AXIS2_PLACEMENT_3D('',#222711,#127769,#127770);
#105575=AXIS2_PLACEMENT_3D('',#222712,#127771,#127772);
#105576=AXIS2_PLACEMENT_3D('',#222713,#127773,#127774);
#105577=AXIS2_PLACEMENT_3D('',#222714,#127775,#127776);
#105578=AXIS2_PLACEMENT_3D('',#222715,#127777,#127778);
#105579=AXIS2_PLACEMENT_3D('',#222716,#127779,#127780);
#105580=AXIS2_PLACEMENT_3D('',#222717,#127781,#127782);
#105581=AXIS2_PLACEMENT_3D('',#222718,#127783,#127784);
#105582=AXIS2_PLACEMENT_3D('',#222719,#127785,#127786);
#105583=AXIS2_PLACEMENT_3D('',#222720,#127787,#127788);
#105584=AXIS2_PLACEMENT_3D('',#222721,#127789,#127790);
#105585=AXIS2_PLACEMENT_3D('',#222722,#127791,#127792);
#105586=AXIS2_PLACEMENT_3D('',#222725,#127793,#127794);
#105587=AXIS2_PLACEMENT_3D('',#222729,#127796,#127797);
#105588=AXIS2_PLACEMENT_3D('',#222731,#127798,#127799);
#105589=AXIS2_PLACEMENT_3D('',#222733,#127800,#127801);
#105590=AXIS2_PLACEMENT_3D('',#222735,#127803,#127804);
#105591=AXIS2_PLACEMENT_3D('',#222739,#127806,#127807);
#105592=AXIS2_PLACEMENT_3D('',#222741,#127809,#127810);
#105593=AXIS2_PLACEMENT_3D('',#222744,#127811,#127812);
#105594=AXIS2_PLACEMENT_3D('',#222748,#127814,#127815);
#105595=AXIS2_PLACEMENT_3D('',#222750,#127817,#127818);
#105596=AXIS2_PLACEMENT_3D('',#222753,#127819,#127820);
#105597=AXIS2_PLACEMENT_3D('',#222757,#127822,#127823);
#105598=AXIS2_PLACEMENT_3D('',#222759,#127824,#127825);
#105599=AXIS2_PLACEMENT_3D('',#222761,#127826,#127827);
#105600=AXIS2_PLACEMENT_3D('',#222763,#127829,#127830);
#105601=AXIS2_PLACEMENT_3D('',#222767,#127832,#127833);
#105602=AXIS2_PLACEMENT_3D('',#222769,#127835,#127836);
#105603=AXIS2_PLACEMENT_3D('',#222770,#127837,#127838);
#105604=AXIS2_PLACEMENT_3D('',#222771,#127839,#127840);
#105605=AXIS2_PLACEMENT_3D('',#222772,#127841,#127842);
#105606=AXIS2_PLACEMENT_3D('',#222773,#127843,#127844);
#105607=AXIS2_PLACEMENT_3D('',#222774,#127845,#127846);
#105608=AXIS2_PLACEMENT_3D('',#222775,#127847,#127848);
#105609=AXIS2_PLACEMENT_3D('',#222776,#127849,#127850);
#105610=AXIS2_PLACEMENT_3D('',#222777,#127851,#127852);
#105611=AXIS2_PLACEMENT_3D('',#222778,#127853,#127854);
#105612=AXIS2_PLACEMENT_3D('',#222779,#127855,#127856);
#105613=AXIS2_PLACEMENT_3D('',#222780,#127857,#127858);
#105614=AXIS2_PLACEMENT_3D('',#222781,#127859,#127860);
#105615=AXIS2_PLACEMENT_3D('',#222784,#127861,#127862);
#105616=AXIS2_PLACEMENT_3D('',#222788,#127864,#127865);
#105617=AXIS2_PLACEMENT_3D('',#222790,#127866,#127867);
#105618=AXIS2_PLACEMENT_3D('',#222792,#127868,#127869);
#105619=AXIS2_PLACEMENT_3D('',#222794,#127871,#127872);
#105620=AXIS2_PLACEMENT_3D('',#222798,#127874,#127875);
#105621=AXIS2_PLACEMENT_3D('',#222800,#127877,#127878);
#105622=AXIS2_PLACEMENT_3D('',#222803,#127879,#127880);
#105623=AXIS2_PLACEMENT_3D('',#222807,#127882,#127883);
#105624=AXIS2_PLACEMENT_3D('',#222809,#127885,#127886);
#105625=AXIS2_PLACEMENT_3D('',#222812,#127887,#127888);
#105626=AXIS2_PLACEMENT_3D('',#222816,#127890,#127891);
#105627=AXIS2_PLACEMENT_3D('',#222818,#127892,#127893);
#105628=AXIS2_PLACEMENT_3D('',#222820,#127894,#127895);
#105629=AXIS2_PLACEMENT_3D('',#222822,#127897,#127898);
#105630=AXIS2_PLACEMENT_3D('',#222826,#127900,#127901);
#105631=AXIS2_PLACEMENT_3D('',#222828,#127903,#127904);
#105632=AXIS2_PLACEMENT_3D('',#222829,#127905,#127906);
#105633=AXIS2_PLACEMENT_3D('',#222830,#127907,#127908);
#105634=AXIS2_PLACEMENT_3D('',#222831,#127909,#127910);
#105635=AXIS2_PLACEMENT_3D('',#222832,#127911,#127912);
#105636=AXIS2_PLACEMENT_3D('',#222833,#127913,#127914);
#105637=AXIS2_PLACEMENT_3D('',#222834,#127915,#127916);
#105638=AXIS2_PLACEMENT_3D('',#222835,#127917,#127918);
#105639=AXIS2_PLACEMENT_3D('',#222836,#127919,#127920);
#105640=AXIS2_PLACEMENT_3D('',#222837,#127921,#127922);
#105641=AXIS2_PLACEMENT_3D('',#222838,#127923,#127924);
#105642=AXIS2_PLACEMENT_3D('',#222839,#127925,#127926);
#105643=AXIS2_PLACEMENT_3D('',#222840,#127927,#127928);
#105644=AXIS2_PLACEMENT_3D('',#222843,#127929,#127930);
#105645=AXIS2_PLACEMENT_3D('',#222847,#127932,#127933);
#105646=AXIS2_PLACEMENT_3D('',#222849,#127934,#127935);
#105647=AXIS2_PLACEMENT_3D('',#222851,#127936,#127937);
#105648=AXIS2_PLACEMENT_3D('',#222853,#127939,#127940);
#105649=AXIS2_PLACEMENT_3D('',#222857,#127942,#127943);
#105650=AXIS2_PLACEMENT_3D('',#222859,#127945,#127946);
#105651=AXIS2_PLACEMENT_3D('',#222862,#127947,#127948);
#105652=AXIS2_PLACEMENT_3D('',#222866,#127950,#127951);
#105653=AXIS2_PLACEMENT_3D('',#222868,#127953,#127954);
#105654=AXIS2_PLACEMENT_3D('',#222871,#127955,#127956);
#105655=AXIS2_PLACEMENT_3D('',#222875,#127958,#127959);
#105656=AXIS2_PLACEMENT_3D('',#222877,#127960,#127961);
#105657=AXIS2_PLACEMENT_3D('',#222879,#127962,#127963);
#105658=AXIS2_PLACEMENT_3D('',#222881,#127965,#127966);
#105659=AXIS2_PLACEMENT_3D('',#222885,#127968,#127969);
#105660=AXIS2_PLACEMENT_3D('',#222887,#127971,#127972);
#105661=AXIS2_PLACEMENT_3D('',#222888,#127973,#127974);
#105662=AXIS2_PLACEMENT_3D('',#222889,#127975,#127976);
#105663=AXIS2_PLACEMENT_3D('',#222890,#127977,#127978);
#105664=AXIS2_PLACEMENT_3D('',#222891,#127979,#127980);
#105665=AXIS2_PLACEMENT_3D('',#222892,#127981,#127982);
#105666=AXIS2_PLACEMENT_3D('',#222893,#127983,#127984);
#105667=AXIS2_PLACEMENT_3D('',#222894,#127985,#127986);
#105668=AXIS2_PLACEMENT_3D('',#222895,#127987,#127988);
#105669=AXIS2_PLACEMENT_3D('',#222896,#127989,#127990);
#105670=AXIS2_PLACEMENT_3D('',#222897,#127991,#127992);
#105671=AXIS2_PLACEMENT_3D('',#222898,#127993,#127994);
#105672=AXIS2_PLACEMENT_3D('',#222899,#127995,#127996);
#105673=AXIS2_PLACEMENT_3D('',#222902,#127997,#127998);
#105674=AXIS2_PLACEMENT_3D('',#222906,#128000,#128001);
#105675=AXIS2_PLACEMENT_3D('',#222908,#128002,#128003);
#105676=AXIS2_PLACEMENT_3D('',#222910,#128004,#128005);
#105677=AXIS2_PLACEMENT_3D('',#222912,#128007,#128008);
#105678=AXIS2_PLACEMENT_3D('',#222916,#128010,#128011);
#105679=AXIS2_PLACEMENT_3D('',#222918,#128013,#128014);
#105680=AXIS2_PLACEMENT_3D('',#222921,#128015,#128016);
#105681=AXIS2_PLACEMENT_3D('',#222925,#128018,#128019);
#105682=AXIS2_PLACEMENT_3D('',#222927,#128021,#128022);
#105683=AXIS2_PLACEMENT_3D('',#222930,#128023,#128024);
#105684=AXIS2_PLACEMENT_3D('',#222934,#128026,#128027);
#105685=AXIS2_PLACEMENT_3D('',#222936,#128028,#128029);
#105686=AXIS2_PLACEMENT_3D('',#222938,#128030,#128031);
#105687=AXIS2_PLACEMENT_3D('',#222940,#128033,#128034);
#105688=AXIS2_PLACEMENT_3D('',#222944,#128036,#128037);
#105689=AXIS2_PLACEMENT_3D('',#222946,#128039,#128040);
#105690=AXIS2_PLACEMENT_3D('',#222947,#128041,#128042);
#105691=AXIS2_PLACEMENT_3D('',#222948,#128043,#128044);
#105692=AXIS2_PLACEMENT_3D('',#222949,#128045,#128046);
#105693=AXIS2_PLACEMENT_3D('',#222950,#128047,#128048);
#105694=AXIS2_PLACEMENT_3D('',#222951,#128049,#128050);
#105695=AXIS2_PLACEMENT_3D('',#222952,#128051,#128052);
#105696=AXIS2_PLACEMENT_3D('',#222953,#128053,#128054);
#105697=AXIS2_PLACEMENT_3D('',#222954,#128055,#128056);
#105698=AXIS2_PLACEMENT_3D('',#222955,#128057,#128058);
#105699=AXIS2_PLACEMENT_3D('',#222956,#128059,#128060);
#105700=AXIS2_PLACEMENT_3D('',#222957,#128061,#128062);
#105701=AXIS2_PLACEMENT_3D('',#222958,#128063,#128064);
#105702=AXIS2_PLACEMENT_3D('',#222961,#128065,#128066);
#105703=AXIS2_PLACEMENT_3D('',#222965,#128068,#128069);
#105704=AXIS2_PLACEMENT_3D('',#222967,#128070,#128071);
#105705=AXIS2_PLACEMENT_3D('',#222969,#128072,#128073);
#105706=AXIS2_PLACEMENT_3D('',#222971,#128075,#128076);
#105707=AXIS2_PLACEMENT_3D('',#222975,#128078,#128079);
#105708=AXIS2_PLACEMENT_3D('',#222977,#128081,#128082);
#105709=AXIS2_PLACEMENT_3D('',#222980,#128083,#128084);
#105710=AXIS2_PLACEMENT_3D('',#222984,#128086,#128087);
#105711=AXIS2_PLACEMENT_3D('',#222986,#128089,#128090);
#105712=AXIS2_PLACEMENT_3D('',#222989,#128091,#128092);
#105713=AXIS2_PLACEMENT_3D('',#222993,#128094,#128095);
#105714=AXIS2_PLACEMENT_3D('',#222995,#128096,#128097);
#105715=AXIS2_PLACEMENT_3D('',#222997,#128098,#128099);
#105716=AXIS2_PLACEMENT_3D('',#222999,#128101,#128102);
#105717=AXIS2_PLACEMENT_3D('',#223003,#128104,#128105);
#105718=AXIS2_PLACEMENT_3D('',#223005,#128107,#128108);
#105719=AXIS2_PLACEMENT_3D('',#223006,#128109,#128110);
#105720=AXIS2_PLACEMENT_3D('',#223007,#128111,#128112);
#105721=AXIS2_PLACEMENT_3D('',#223008,#128113,#128114);
#105722=AXIS2_PLACEMENT_3D('',#223009,#128115,#128116);
#105723=AXIS2_PLACEMENT_3D('',#223010,#128117,#128118);
#105724=AXIS2_PLACEMENT_3D('',#223011,#128119,#128120);
#105725=AXIS2_PLACEMENT_3D('',#223012,#128121,#128122);
#105726=AXIS2_PLACEMENT_3D('',#223013,#128123,#128124);
#105727=AXIS2_PLACEMENT_3D('',#223014,#128125,#128126);
#105728=AXIS2_PLACEMENT_3D('',#223015,#128127,#128128);
#105729=AXIS2_PLACEMENT_3D('',#223016,#128129,#128130);
#105730=AXIS2_PLACEMENT_3D('',#223017,#128131,#128132);
#105731=AXIS2_PLACEMENT_3D('',#223020,#128133,#128134);
#105732=AXIS2_PLACEMENT_3D('',#223024,#128136,#128137);
#105733=AXIS2_PLACEMENT_3D('',#223026,#128138,#128139);
#105734=AXIS2_PLACEMENT_3D('',#223028,#128140,#128141);
#105735=AXIS2_PLACEMENT_3D('',#223030,#128143,#128144);
#105736=AXIS2_PLACEMENT_3D('',#223034,#128146,#128147);
#105737=AXIS2_PLACEMENT_3D('',#223036,#128149,#128150);
#105738=AXIS2_PLACEMENT_3D('',#223039,#128151,#128152);
#105739=AXIS2_PLACEMENT_3D('',#223043,#128154,#128155);
#105740=AXIS2_PLACEMENT_3D('',#223045,#128157,#128158);
#105741=AXIS2_PLACEMENT_3D('',#223048,#128159,#128160);
#105742=AXIS2_PLACEMENT_3D('',#223052,#128162,#128163);
#105743=AXIS2_PLACEMENT_3D('',#223054,#128164,#128165);
#105744=AXIS2_PLACEMENT_3D('',#223056,#128166,#128167);
#105745=AXIS2_PLACEMENT_3D('',#223058,#128169,#128170);
#105746=AXIS2_PLACEMENT_3D('',#223062,#128172,#128173);
#105747=AXIS2_PLACEMENT_3D('',#223064,#128175,#128176);
#105748=AXIS2_PLACEMENT_3D('',#223065,#128177,#128178);
#105749=AXIS2_PLACEMENT_3D('',#223066,#128179,#128180);
#105750=AXIS2_PLACEMENT_3D('',#223067,#128181,#128182);
#105751=AXIS2_PLACEMENT_3D('',#223068,#128183,#128184);
#105752=AXIS2_PLACEMENT_3D('',#223069,#128185,#128186);
#105753=AXIS2_PLACEMENT_3D('',#223070,#128187,#128188);
#105754=AXIS2_PLACEMENT_3D('',#223071,#128189,#128190);
#105755=AXIS2_PLACEMENT_3D('',#223072,#128191,#128192);
#105756=AXIS2_PLACEMENT_3D('',#223073,#128193,#128194);
#105757=AXIS2_PLACEMENT_3D('',#223074,#128195,#128196);
#105758=AXIS2_PLACEMENT_3D('',#223075,#128197,#128198);
#105759=AXIS2_PLACEMENT_3D('',#223076,#128199,#128200);
#105760=AXIS2_PLACEMENT_3D('',#223079,#128201,#128202);
#105761=AXIS2_PLACEMENT_3D('',#223083,#128204,#128205);
#105762=AXIS2_PLACEMENT_3D('',#223085,#128206,#128207);
#105763=AXIS2_PLACEMENT_3D('',#223087,#128208,#128209);
#105764=AXIS2_PLACEMENT_3D('',#223089,#128211,#128212);
#105765=AXIS2_PLACEMENT_3D('',#223093,#128214,#128215);
#105766=AXIS2_PLACEMENT_3D('',#223095,#128217,#128218);
#105767=AXIS2_PLACEMENT_3D('',#223098,#128219,#128220);
#105768=AXIS2_PLACEMENT_3D('',#223102,#128222,#128223);
#105769=AXIS2_PLACEMENT_3D('',#223104,#128225,#128226);
#105770=AXIS2_PLACEMENT_3D('',#223107,#128227,#128228);
#105771=AXIS2_PLACEMENT_3D('',#223111,#128230,#128231);
#105772=AXIS2_PLACEMENT_3D('',#223113,#128232,#128233);
#105773=AXIS2_PLACEMENT_3D('',#223115,#128234,#128235);
#105774=AXIS2_PLACEMENT_3D('',#223117,#128237,#128238);
#105775=AXIS2_PLACEMENT_3D('',#223121,#128240,#128241);
#105776=AXIS2_PLACEMENT_3D('',#223123,#128243,#128244);
#105777=AXIS2_PLACEMENT_3D('',#223124,#128245,#128246);
#105778=AXIS2_PLACEMENT_3D('',#223125,#128247,#128248);
#105779=AXIS2_PLACEMENT_3D('',#223126,#128249,#128250);
#105780=AXIS2_PLACEMENT_3D('',#223127,#128251,#128252);
#105781=AXIS2_PLACEMENT_3D('',#223128,#128253,#128254);
#105782=AXIS2_PLACEMENT_3D('',#223129,#128255,#128256);
#105783=AXIS2_PLACEMENT_3D('',#223130,#128257,#128258);
#105784=AXIS2_PLACEMENT_3D('',#223131,#128259,#128260);
#105785=AXIS2_PLACEMENT_3D('',#223132,#128261,#128262);
#105786=AXIS2_PLACEMENT_3D('',#223133,#128263,#128264);
#105787=AXIS2_PLACEMENT_3D('',#223134,#128265,#128266);
#105788=AXIS2_PLACEMENT_3D('',#223135,#128267,#128268);
#105789=AXIS2_PLACEMENT_3D('',#223138,#128269,#128270);
#105790=AXIS2_PLACEMENT_3D('',#223142,#128272,#128273);
#105791=AXIS2_PLACEMENT_3D('',#223144,#128274,#128275);
#105792=AXIS2_PLACEMENT_3D('',#223146,#128276,#128277);
#105793=AXIS2_PLACEMENT_3D('',#223148,#128279,#128280);
#105794=AXIS2_PLACEMENT_3D('',#223152,#128282,#128283);
#105795=AXIS2_PLACEMENT_3D('',#223154,#128285,#128286);
#105796=AXIS2_PLACEMENT_3D('',#223157,#128287,#128288);
#105797=AXIS2_PLACEMENT_3D('',#223161,#128290,#128291);
#105798=AXIS2_PLACEMENT_3D('',#223163,#128293,#128294);
#105799=AXIS2_PLACEMENT_3D('',#223166,#128295,#128296);
#105800=AXIS2_PLACEMENT_3D('',#223170,#128298,#128299);
#105801=AXIS2_PLACEMENT_3D('',#223172,#128300,#128301);
#105802=AXIS2_PLACEMENT_3D('',#223174,#128302,#128303);
#105803=AXIS2_PLACEMENT_3D('',#223176,#128305,#128306);
#105804=AXIS2_PLACEMENT_3D('',#223180,#128308,#128309);
#105805=AXIS2_PLACEMENT_3D('',#223182,#128311,#128312);
#105806=AXIS2_PLACEMENT_3D('',#223183,#128313,#128314);
#105807=AXIS2_PLACEMENT_3D('',#223184,#128315,#128316);
#105808=AXIS2_PLACEMENT_3D('',#223185,#128317,#128318);
#105809=AXIS2_PLACEMENT_3D('',#223186,#128319,#128320);
#105810=AXIS2_PLACEMENT_3D('',#223187,#128321,#128322);
#105811=AXIS2_PLACEMENT_3D('',#223188,#128323,#128324);
#105812=AXIS2_PLACEMENT_3D('',#223189,#128325,#128326);
#105813=AXIS2_PLACEMENT_3D('',#223190,#128327,#128328);
#105814=AXIS2_PLACEMENT_3D('',#223191,#128329,#128330);
#105815=AXIS2_PLACEMENT_3D('',#223192,#128331,#128332);
#105816=AXIS2_PLACEMENT_3D('',#223193,#128333,#128334);
#105817=AXIS2_PLACEMENT_3D('',#223194,#128335,#128336);
#105818=AXIS2_PLACEMENT_3D('',#223197,#128337,#128338);
#105819=AXIS2_PLACEMENT_3D('',#223201,#128340,#128341);
#105820=AXIS2_PLACEMENT_3D('',#223203,#128342,#128343);
#105821=AXIS2_PLACEMENT_3D('',#223205,#128344,#128345);
#105822=AXIS2_PLACEMENT_3D('',#223207,#128347,#128348);
#105823=AXIS2_PLACEMENT_3D('',#223211,#128350,#128351);
#105824=AXIS2_PLACEMENT_3D('',#223213,#128353,#128354);
#105825=AXIS2_PLACEMENT_3D('',#223216,#128355,#128356);
#105826=AXIS2_PLACEMENT_3D('',#223220,#128358,#128359);
#105827=AXIS2_PLACEMENT_3D('',#223222,#128361,#128362);
#105828=AXIS2_PLACEMENT_3D('',#223225,#128363,#128364);
#105829=AXIS2_PLACEMENT_3D('',#223229,#128366,#128367);
#105830=AXIS2_PLACEMENT_3D('',#223231,#128368,#128369);
#105831=AXIS2_PLACEMENT_3D('',#223233,#128370,#128371);
#105832=AXIS2_PLACEMENT_3D('',#223235,#128373,#128374);
#105833=AXIS2_PLACEMENT_3D('',#223239,#128376,#128377);
#105834=AXIS2_PLACEMENT_3D('',#223241,#128379,#128380);
#105835=AXIS2_PLACEMENT_3D('',#223242,#128381,#128382);
#105836=AXIS2_PLACEMENT_3D('',#223243,#128383,#128384);
#105837=AXIS2_PLACEMENT_3D('',#223244,#128385,#128386);
#105838=AXIS2_PLACEMENT_3D('',#223245,#128387,#128388);
#105839=AXIS2_PLACEMENT_3D('',#223246,#128389,#128390);
#105840=AXIS2_PLACEMENT_3D('',#223247,#128391,#128392);
#105841=AXIS2_PLACEMENT_3D('',#223248,#128393,#128394);
#105842=AXIS2_PLACEMENT_3D('',#223249,#128395,#128396);
#105843=AXIS2_PLACEMENT_3D('',#223250,#128397,#128398);
#105844=AXIS2_PLACEMENT_3D('',#223251,#128399,#128400);
#105845=AXIS2_PLACEMENT_3D('',#223252,#128401,#128402);
#105846=AXIS2_PLACEMENT_3D('',#223253,#128403,#128404);
#105847=AXIS2_PLACEMENT_3D('',#223256,#128405,#128406);
#105848=AXIS2_PLACEMENT_3D('',#223260,#128408,#128409);
#105849=AXIS2_PLACEMENT_3D('',#223262,#128410,#128411);
#105850=AXIS2_PLACEMENT_3D('',#223264,#128412,#128413);
#105851=AXIS2_PLACEMENT_3D('',#223266,#128415,#128416);
#105852=AXIS2_PLACEMENT_3D('',#223270,#128418,#128419);
#105853=AXIS2_PLACEMENT_3D('',#223272,#128421,#128422);
#105854=AXIS2_PLACEMENT_3D('',#223275,#128423,#128424);
#105855=AXIS2_PLACEMENT_3D('',#223279,#128426,#128427);
#105856=AXIS2_PLACEMENT_3D('',#223281,#128429,#128430);
#105857=AXIS2_PLACEMENT_3D('',#223284,#128431,#128432);
#105858=AXIS2_PLACEMENT_3D('',#223288,#128434,#128435);
#105859=AXIS2_PLACEMENT_3D('',#223290,#128436,#128437);
#105860=AXIS2_PLACEMENT_3D('',#223292,#128438,#128439);
#105861=AXIS2_PLACEMENT_3D('',#223294,#128441,#128442);
#105862=AXIS2_PLACEMENT_3D('',#223298,#128444,#128445);
#105863=AXIS2_PLACEMENT_3D('',#223300,#128447,#128448);
#105864=AXIS2_PLACEMENT_3D('',#223301,#128449,#128450);
#105865=AXIS2_PLACEMENT_3D('',#223302,#128451,#128452);
#105866=AXIS2_PLACEMENT_3D('',#223303,#128453,#128454);
#105867=AXIS2_PLACEMENT_3D('',#223304,#128455,#128456);
#105868=AXIS2_PLACEMENT_3D('',#223305,#128457,#128458);
#105869=AXIS2_PLACEMENT_3D('',#223306,#128459,#128460);
#105870=AXIS2_PLACEMENT_3D('',#223307,#128461,#128462);
#105871=AXIS2_PLACEMENT_3D('',#223308,#128463,#128464);
#105872=AXIS2_PLACEMENT_3D('',#223309,#128465,#128466);
#105873=AXIS2_PLACEMENT_3D('',#223310,#128467,#128468);
#105874=AXIS2_PLACEMENT_3D('',#223311,#128469,#128470);
#105875=AXIS2_PLACEMENT_3D('',#223312,#128471,#128472);
#105876=AXIS2_PLACEMENT_3D('',#223315,#128473,#128474);
#105877=AXIS2_PLACEMENT_3D('',#223319,#128476,#128477);
#105878=AXIS2_PLACEMENT_3D('',#223321,#128478,#128479);
#105879=AXIS2_PLACEMENT_3D('',#223323,#128480,#128481);
#105880=AXIS2_PLACEMENT_3D('',#223325,#128483,#128484);
#105881=AXIS2_PLACEMENT_3D('',#223329,#128486,#128487);
#105882=AXIS2_PLACEMENT_3D('',#223331,#128489,#128490);
#105883=AXIS2_PLACEMENT_3D('',#223334,#128491,#128492);
#105884=AXIS2_PLACEMENT_3D('',#223338,#128494,#128495);
#105885=AXIS2_PLACEMENT_3D('',#223340,#128497,#128498);
#105886=AXIS2_PLACEMENT_3D('',#223343,#128499,#128500);
#105887=AXIS2_PLACEMENT_3D('',#223347,#128502,#128503);
#105888=AXIS2_PLACEMENT_3D('',#223349,#128504,#128505);
#105889=AXIS2_PLACEMENT_3D('',#223351,#128506,#128507);
#105890=AXIS2_PLACEMENT_3D('',#223353,#128509,#128510);
#105891=AXIS2_PLACEMENT_3D('',#223357,#128512,#128513);
#105892=AXIS2_PLACEMENT_3D('',#223359,#128515,#128516);
#105893=AXIS2_PLACEMENT_3D('',#223360,#128517,#128518);
#105894=AXIS2_PLACEMENT_3D('',#223361,#128519,#128520);
#105895=AXIS2_PLACEMENT_3D('',#223362,#128521,#128522);
#105896=AXIS2_PLACEMENT_3D('',#223363,#128523,#128524);
#105897=AXIS2_PLACEMENT_3D('',#223364,#128525,#128526);
#105898=AXIS2_PLACEMENT_3D('',#223365,#128527,#128528);
#105899=AXIS2_PLACEMENT_3D('',#223366,#128529,#128530);
#105900=AXIS2_PLACEMENT_3D('',#223367,#128531,#128532);
#105901=AXIS2_PLACEMENT_3D('',#223368,#128533,#128534);
#105902=AXIS2_PLACEMENT_3D('',#223369,#128535,#128536);
#105903=AXIS2_PLACEMENT_3D('',#223370,#128537,#128538);
#105904=AXIS2_PLACEMENT_3D('',#223371,#128539,#128540);
#105905=AXIS2_PLACEMENT_3D('',#223374,#128541,#128542);
#105906=AXIS2_PLACEMENT_3D('',#223378,#128544,#128545);
#105907=AXIS2_PLACEMENT_3D('',#223380,#128546,#128547);
#105908=AXIS2_PLACEMENT_3D('',#223382,#128548,#128549);
#105909=AXIS2_PLACEMENT_3D('',#223384,#128551,#128552);
#105910=AXIS2_PLACEMENT_3D('',#223388,#128554,#128555);
#105911=AXIS2_PLACEMENT_3D('',#223390,#128557,#128558);
#105912=AXIS2_PLACEMENT_3D('',#223393,#128559,#128560);
#105913=AXIS2_PLACEMENT_3D('',#223397,#128562,#128563);
#105914=AXIS2_PLACEMENT_3D('',#223399,#128565,#128566);
#105915=AXIS2_PLACEMENT_3D('',#223402,#128567,#128568);
#105916=AXIS2_PLACEMENT_3D('',#223406,#128570,#128571);
#105917=AXIS2_PLACEMENT_3D('',#223408,#128572,#128573);
#105918=AXIS2_PLACEMENT_3D('',#223410,#128574,#128575);
#105919=AXIS2_PLACEMENT_3D('',#223412,#128577,#128578);
#105920=AXIS2_PLACEMENT_3D('',#223416,#128580,#128581);
#105921=AXIS2_PLACEMENT_3D('',#223418,#128583,#128584);
#105922=AXIS2_PLACEMENT_3D('',#223419,#128585,#128586);
#105923=AXIS2_PLACEMENT_3D('',#223420,#128587,#128588);
#105924=AXIS2_PLACEMENT_3D('',#223421,#128589,#128590);
#105925=AXIS2_PLACEMENT_3D('',#223422,#128591,#128592);
#105926=AXIS2_PLACEMENT_3D('',#223423,#128593,#128594);
#105927=AXIS2_PLACEMENT_3D('',#223424,#128595,#128596);
#105928=AXIS2_PLACEMENT_3D('',#223425,#128597,#128598);
#105929=AXIS2_PLACEMENT_3D('',#223426,#128599,#128600);
#105930=AXIS2_PLACEMENT_3D('',#223427,#128601,#128602);
#105931=AXIS2_PLACEMENT_3D('',#223428,#128603,#128604);
#105932=AXIS2_PLACEMENT_3D('',#223429,#128605,#128606);
#105933=AXIS2_PLACEMENT_3D('',#223430,#128607,#128608);
#105934=AXIS2_PLACEMENT_3D('',#223433,#128609,#128610);
#105935=AXIS2_PLACEMENT_3D('',#223437,#128612,#128613);
#105936=AXIS2_PLACEMENT_3D('',#223439,#128614,#128615);
#105937=AXIS2_PLACEMENT_3D('',#223441,#128616,#128617);
#105938=AXIS2_PLACEMENT_3D('',#223443,#128619,#128620);
#105939=AXIS2_PLACEMENT_3D('',#223447,#128622,#128623);
#105940=AXIS2_PLACEMENT_3D('',#223449,#128625,#128626);
#105941=AXIS2_PLACEMENT_3D('',#223452,#128627,#128628);
#105942=AXIS2_PLACEMENT_3D('',#223456,#128630,#128631);
#105943=AXIS2_PLACEMENT_3D('',#223458,#128633,#128634);
#105944=AXIS2_PLACEMENT_3D('',#223461,#128635,#128636);
#105945=AXIS2_PLACEMENT_3D('',#223465,#128638,#128639);
#105946=AXIS2_PLACEMENT_3D('',#223467,#128640,#128641);
#105947=AXIS2_PLACEMENT_3D('',#223469,#128642,#128643);
#105948=AXIS2_PLACEMENT_3D('',#223471,#128645,#128646);
#105949=AXIS2_PLACEMENT_3D('',#223475,#128648,#128649);
#105950=AXIS2_PLACEMENT_3D('',#223477,#128651,#128652);
#105951=AXIS2_PLACEMENT_3D('',#223478,#128653,#128654);
#105952=AXIS2_PLACEMENT_3D('',#223479,#128655,#128656);
#105953=AXIS2_PLACEMENT_3D('',#223480,#128657,#128658);
#105954=AXIS2_PLACEMENT_3D('',#223481,#128659,#128660);
#105955=AXIS2_PLACEMENT_3D('',#223482,#128661,#128662);
#105956=AXIS2_PLACEMENT_3D('',#223483,#128663,#128664);
#105957=AXIS2_PLACEMENT_3D('',#223484,#128665,#128666);
#105958=AXIS2_PLACEMENT_3D('',#223485,#128667,#128668);
#105959=AXIS2_PLACEMENT_3D('',#223486,#128669,#128670);
#105960=AXIS2_PLACEMENT_3D('',#223487,#128671,#128672);
#105961=AXIS2_PLACEMENT_3D('',#223488,#128673,#128674);
#105962=AXIS2_PLACEMENT_3D('',#223489,#128675,#128676);
#105963=AXIS2_PLACEMENT_3D('',#223492,#128677,#128678);
#105964=AXIS2_PLACEMENT_3D('',#223496,#128680,#128681);
#105965=AXIS2_PLACEMENT_3D('',#223498,#128682,#128683);
#105966=AXIS2_PLACEMENT_3D('',#223500,#128684,#128685);
#105967=AXIS2_PLACEMENT_3D('',#223502,#128687,#128688);
#105968=AXIS2_PLACEMENT_3D('',#223506,#128690,#128691);
#105969=AXIS2_PLACEMENT_3D('',#223508,#128693,#128694);
#105970=AXIS2_PLACEMENT_3D('',#223511,#128695,#128696);
#105971=AXIS2_PLACEMENT_3D('',#223515,#128698,#128699);
#105972=AXIS2_PLACEMENT_3D('',#223517,#128701,#128702);
#105973=AXIS2_PLACEMENT_3D('',#223520,#128703,#128704);
#105974=AXIS2_PLACEMENT_3D('',#223524,#128706,#128707);
#105975=AXIS2_PLACEMENT_3D('',#223526,#128708,#128709);
#105976=AXIS2_PLACEMENT_3D('',#223528,#128710,#128711);
#105977=AXIS2_PLACEMENT_3D('',#223530,#128713,#128714);
#105978=AXIS2_PLACEMENT_3D('',#223534,#128716,#128717);
#105979=AXIS2_PLACEMENT_3D('',#223536,#128719,#128720);
#105980=AXIS2_PLACEMENT_3D('',#223537,#128721,#128722);
#105981=AXIS2_PLACEMENT_3D('',#223538,#128723,#128724);
#105982=AXIS2_PLACEMENT_3D('',#223539,#128725,#128726);
#105983=AXIS2_PLACEMENT_3D('',#223540,#128727,#128728);
#105984=AXIS2_PLACEMENT_3D('',#223541,#128729,#128730);
#105985=AXIS2_PLACEMENT_3D('',#223542,#128731,#128732);
#105986=AXIS2_PLACEMENT_3D('',#223543,#128733,#128734);
#105987=AXIS2_PLACEMENT_3D('',#223544,#128735,#128736);
#105988=AXIS2_PLACEMENT_3D('',#223545,#128737,#128738);
#105989=AXIS2_PLACEMENT_3D('',#223546,#128739,#128740);
#105990=AXIS2_PLACEMENT_3D('',#223547,#128741,#128742);
#105991=AXIS2_PLACEMENT_3D('',#223548,#128743,#128744);
#105992=AXIS2_PLACEMENT_3D('',#223551,#128745,#128746);
#105993=AXIS2_PLACEMENT_3D('',#223555,#128748,#128749);
#105994=AXIS2_PLACEMENT_3D('',#223557,#128750,#128751);
#105995=AXIS2_PLACEMENT_3D('',#223559,#128752,#128753);
#105996=AXIS2_PLACEMENT_3D('',#223561,#128755,#128756);
#105997=AXIS2_PLACEMENT_3D('',#223565,#128758,#128759);
#105998=AXIS2_PLACEMENT_3D('',#223567,#128761,#128762);
#105999=AXIS2_PLACEMENT_3D('',#223570,#128763,#128764);
#106000=AXIS2_PLACEMENT_3D('',#223574,#128766,#128767);
#106001=AXIS2_PLACEMENT_3D('',#223576,#128769,#128770);
#106002=AXIS2_PLACEMENT_3D('',#223579,#128771,#128772);
#106003=AXIS2_PLACEMENT_3D('',#223583,#128774,#128775);
#106004=AXIS2_PLACEMENT_3D('',#223585,#128776,#128777);
#106005=AXIS2_PLACEMENT_3D('',#223587,#128778,#128779);
#106006=AXIS2_PLACEMENT_3D('',#223589,#128781,#128782);
#106007=AXIS2_PLACEMENT_3D('',#223593,#128784,#128785);
#106008=AXIS2_PLACEMENT_3D('',#223595,#128787,#128788);
#106009=AXIS2_PLACEMENT_3D('',#223596,#128789,#128790);
#106010=AXIS2_PLACEMENT_3D('',#223597,#128791,#128792);
#106011=AXIS2_PLACEMENT_3D('',#223598,#128793,#128794);
#106012=AXIS2_PLACEMENT_3D('',#223599,#128795,#128796);
#106013=AXIS2_PLACEMENT_3D('',#223600,#128797,#128798);
#106014=AXIS2_PLACEMENT_3D('',#223601,#128799,#128800);
#106015=AXIS2_PLACEMENT_3D('',#223602,#128801,#128802);
#106016=AXIS2_PLACEMENT_3D('',#223603,#128803,#128804);
#106017=AXIS2_PLACEMENT_3D('',#223604,#128805,#128806);
#106018=AXIS2_PLACEMENT_3D('',#223605,#128807,#128808);
#106019=AXIS2_PLACEMENT_3D('',#223606,#128809,#128810);
#106020=AXIS2_PLACEMENT_3D('',#223607,#128811,#128812);
#106021=AXIS2_PLACEMENT_3D('',#223610,#128813,#128814);
#106022=AXIS2_PLACEMENT_3D('',#223614,#128816,#128817);
#106023=AXIS2_PLACEMENT_3D('',#223616,#128818,#128819);
#106024=AXIS2_PLACEMENT_3D('',#223618,#128820,#128821);
#106025=AXIS2_PLACEMENT_3D('',#223620,#128823,#128824);
#106026=AXIS2_PLACEMENT_3D('',#223624,#128826,#128827);
#106027=AXIS2_PLACEMENT_3D('',#223626,#128829,#128830);
#106028=AXIS2_PLACEMENT_3D('',#223629,#128831,#128832);
#106029=AXIS2_PLACEMENT_3D('',#223633,#128834,#128835);
#106030=AXIS2_PLACEMENT_3D('',#223635,#128837,#128838);
#106031=AXIS2_PLACEMENT_3D('',#223638,#128839,#128840);
#106032=AXIS2_PLACEMENT_3D('',#223642,#128842,#128843);
#106033=AXIS2_PLACEMENT_3D('',#223644,#128844,#128845);
#106034=AXIS2_PLACEMENT_3D('',#223646,#128846,#128847);
#106035=AXIS2_PLACEMENT_3D('',#223648,#128849,#128850);
#106036=AXIS2_PLACEMENT_3D('',#223652,#128852,#128853);
#106037=AXIS2_PLACEMENT_3D('',#223654,#128855,#128856);
#106038=AXIS2_PLACEMENT_3D('',#223655,#128857,#128858);
#106039=AXIS2_PLACEMENT_3D('',#223656,#128859,#128860);
#106040=AXIS2_PLACEMENT_3D('',#223657,#128861,#128862);
#106041=AXIS2_PLACEMENT_3D('',#223658,#128863,#128864);
#106042=AXIS2_PLACEMENT_3D('',#223659,#128865,#128866);
#106043=AXIS2_PLACEMENT_3D('',#223660,#128867,#128868);
#106044=AXIS2_PLACEMENT_3D('',#223661,#128869,#128870);
#106045=AXIS2_PLACEMENT_3D('',#223662,#128871,#128872);
#106046=AXIS2_PLACEMENT_3D('',#223663,#128873,#128874);
#106047=AXIS2_PLACEMENT_3D('',#223664,#128875,#128876);
#106048=AXIS2_PLACEMENT_3D('',#223665,#128877,#128878);
#106049=AXIS2_PLACEMENT_3D('',#223666,#128879,#128880);
#106050=AXIS2_PLACEMENT_3D('',#223669,#128881,#128882);
#106051=AXIS2_PLACEMENT_3D('',#223673,#128884,#128885);
#106052=AXIS2_PLACEMENT_3D('',#223675,#128886,#128887);
#106053=AXIS2_PLACEMENT_3D('',#223677,#128888,#128889);
#106054=AXIS2_PLACEMENT_3D('',#223679,#128891,#128892);
#106055=AXIS2_PLACEMENT_3D('',#223683,#128894,#128895);
#106056=AXIS2_PLACEMENT_3D('',#223685,#128897,#128898);
#106057=AXIS2_PLACEMENT_3D('',#223688,#128899,#128900);
#106058=AXIS2_PLACEMENT_3D('',#223692,#128902,#128903);
#106059=AXIS2_PLACEMENT_3D('',#223694,#128905,#128906);
#106060=AXIS2_PLACEMENT_3D('',#223697,#128907,#128908);
#106061=AXIS2_PLACEMENT_3D('',#223701,#128910,#128911);
#106062=AXIS2_PLACEMENT_3D('',#223703,#128912,#128913);
#106063=AXIS2_PLACEMENT_3D('',#223705,#128914,#128915);
#106064=AXIS2_PLACEMENT_3D('',#223707,#128917,#128918);
#106065=AXIS2_PLACEMENT_3D('',#223711,#128920,#128921);
#106066=AXIS2_PLACEMENT_3D('',#223713,#128923,#128924);
#106067=AXIS2_PLACEMENT_3D('',#223714,#128925,#128926);
#106068=AXIS2_PLACEMENT_3D('',#223715,#128927,#128928);
#106069=AXIS2_PLACEMENT_3D('',#223716,#128929,#128930);
#106070=AXIS2_PLACEMENT_3D('',#223717,#128931,#128932);
#106071=AXIS2_PLACEMENT_3D('',#223718,#128933,#128934);
#106072=AXIS2_PLACEMENT_3D('',#223719,#128935,#128936);
#106073=AXIS2_PLACEMENT_3D('',#223720,#128937,#128938);
#106074=AXIS2_PLACEMENT_3D('',#223721,#128939,#128940);
#106075=AXIS2_PLACEMENT_3D('',#223722,#128941,#128942);
#106076=AXIS2_PLACEMENT_3D('',#223723,#128943,#128944);
#106077=AXIS2_PLACEMENT_3D('',#223724,#128945,#128946);
#106078=AXIS2_PLACEMENT_3D('',#223725,#128947,#128948);
#106079=AXIS2_PLACEMENT_3D('',#223728,#128949,#128950);
#106080=AXIS2_PLACEMENT_3D('',#223732,#128952,#128953);
#106081=AXIS2_PLACEMENT_3D('',#223734,#128954,#128955);
#106082=AXIS2_PLACEMENT_3D('',#223736,#128956,#128957);
#106083=AXIS2_PLACEMENT_3D('',#223738,#128959,#128960);
#106084=AXIS2_PLACEMENT_3D('',#223742,#128962,#128963);
#106085=AXIS2_PLACEMENT_3D('',#223744,#128965,#128966);
#106086=AXIS2_PLACEMENT_3D('',#223747,#128967,#128968);
#106087=AXIS2_PLACEMENT_3D('',#223751,#128970,#128971);
#106088=AXIS2_PLACEMENT_3D('',#223753,#128973,#128974);
#106089=AXIS2_PLACEMENT_3D('',#223756,#128975,#128976);
#106090=AXIS2_PLACEMENT_3D('',#223760,#128978,#128979);
#106091=AXIS2_PLACEMENT_3D('',#223762,#128980,#128981);
#106092=AXIS2_PLACEMENT_3D('',#223764,#128982,#128983);
#106093=AXIS2_PLACEMENT_3D('',#223766,#128985,#128986);
#106094=AXIS2_PLACEMENT_3D('',#223770,#128988,#128989);
#106095=AXIS2_PLACEMENT_3D('',#223772,#128991,#128992);
#106096=AXIS2_PLACEMENT_3D('',#223773,#128993,#128994);
#106097=AXIS2_PLACEMENT_3D('',#223774,#128995,#128996);
#106098=AXIS2_PLACEMENT_3D('',#223775,#128997,#128998);
#106099=AXIS2_PLACEMENT_3D('',#223776,#128999,#129000);
#106100=AXIS2_PLACEMENT_3D('',#223777,#129001,#129002);
#106101=AXIS2_PLACEMENT_3D('',#223778,#129003,#129004);
#106102=AXIS2_PLACEMENT_3D('',#223779,#129005,#129006);
#106103=AXIS2_PLACEMENT_3D('',#223780,#129007,#129008);
#106104=AXIS2_PLACEMENT_3D('',#223781,#129009,#129010);
#106105=AXIS2_PLACEMENT_3D('',#223782,#129011,#129012);
#106106=AXIS2_PLACEMENT_3D('',#223783,#129013,#129014);
#106107=AXIS2_PLACEMENT_3D('',#223784,#129015,#129016);
#106108=AXIS2_PLACEMENT_3D('',#223787,#129017,#129018);
#106109=AXIS2_PLACEMENT_3D('',#223791,#129020,#129021);
#106110=AXIS2_PLACEMENT_3D('',#223793,#129022,#129023);
#106111=AXIS2_PLACEMENT_3D('',#223795,#129024,#129025);
#106112=AXIS2_PLACEMENT_3D('',#223797,#129027,#129028);
#106113=AXIS2_PLACEMENT_3D('',#223801,#129030,#129031);
#106114=AXIS2_PLACEMENT_3D('',#223803,#129033,#129034);
#106115=AXIS2_PLACEMENT_3D('',#223806,#129035,#129036);
#106116=AXIS2_PLACEMENT_3D('',#223810,#129038,#129039);
#106117=AXIS2_PLACEMENT_3D('',#223812,#129041,#129042);
#106118=AXIS2_PLACEMENT_3D('',#223815,#129043,#129044);
#106119=AXIS2_PLACEMENT_3D('',#223819,#129046,#129047);
#106120=AXIS2_PLACEMENT_3D('',#223821,#129048,#129049);
#106121=AXIS2_PLACEMENT_3D('',#223823,#129050,#129051);
#106122=AXIS2_PLACEMENT_3D('',#223825,#129053,#129054);
#106123=AXIS2_PLACEMENT_3D('',#223829,#129056,#129057);
#106124=AXIS2_PLACEMENT_3D('',#223831,#129059,#129060);
#106125=AXIS2_PLACEMENT_3D('',#223832,#129061,#129062);
#106126=AXIS2_PLACEMENT_3D('',#223833,#129063,#129064);
#106127=AXIS2_PLACEMENT_3D('',#223834,#129065,#129066);
#106128=AXIS2_PLACEMENT_3D('',#223835,#129067,#129068);
#106129=AXIS2_PLACEMENT_3D('',#223836,#129069,#129070);
#106130=AXIS2_PLACEMENT_3D('',#223837,#129071,#129072);
#106131=AXIS2_PLACEMENT_3D('',#223838,#129073,#129074);
#106132=AXIS2_PLACEMENT_3D('',#223839,#129075,#129076);
#106133=AXIS2_PLACEMENT_3D('',#223840,#129077,#129078);
#106134=AXIS2_PLACEMENT_3D('',#223841,#129079,#129080);
#106135=AXIS2_PLACEMENT_3D('',#223842,#129081,#129082);
#106136=AXIS2_PLACEMENT_3D('',#223843,#129083,#129084);
#106137=AXIS2_PLACEMENT_3D('',#223846,#129085,#129086);
#106138=AXIS2_PLACEMENT_3D('',#223850,#129088,#129089);
#106139=AXIS2_PLACEMENT_3D('',#223852,#129090,#129091);
#106140=AXIS2_PLACEMENT_3D('',#223854,#129092,#129093);
#106141=AXIS2_PLACEMENT_3D('',#223856,#129095,#129096);
#106142=AXIS2_PLACEMENT_3D('',#223860,#129098,#129099);
#106143=AXIS2_PLACEMENT_3D('',#223862,#129101,#129102);
#106144=AXIS2_PLACEMENT_3D('',#223865,#129103,#129104);
#106145=AXIS2_PLACEMENT_3D('',#223869,#129106,#129107);
#106146=AXIS2_PLACEMENT_3D('',#223871,#129109,#129110);
#106147=AXIS2_PLACEMENT_3D('',#223874,#129111,#129112);
#106148=AXIS2_PLACEMENT_3D('',#223878,#129114,#129115);
#106149=AXIS2_PLACEMENT_3D('',#223880,#129116,#129117);
#106150=AXIS2_PLACEMENT_3D('',#223882,#129118,#129119);
#106151=AXIS2_PLACEMENT_3D('',#223884,#129121,#129122);
#106152=AXIS2_PLACEMENT_3D('',#223888,#129124,#129125);
#106153=AXIS2_PLACEMENT_3D('',#223890,#129127,#129128);
#106154=AXIS2_PLACEMENT_3D('',#223891,#129129,#129130);
#106155=AXIS2_PLACEMENT_3D('',#223892,#129131,#129132);
#106156=AXIS2_PLACEMENT_3D('',#223893,#129133,#129134);
#106157=AXIS2_PLACEMENT_3D('',#223894,#129135,#129136);
#106158=AXIS2_PLACEMENT_3D('',#223895,#129137,#129138);
#106159=AXIS2_PLACEMENT_3D('',#223896,#129139,#129140);
#106160=AXIS2_PLACEMENT_3D('',#223897,#129141,#129142);
#106161=AXIS2_PLACEMENT_3D('',#223898,#129143,#129144);
#106162=AXIS2_PLACEMENT_3D('',#223899,#129145,#129146);
#106163=AXIS2_PLACEMENT_3D('',#223900,#129147,#129148);
#106164=AXIS2_PLACEMENT_3D('',#223901,#129149,#129150);
#106165=AXIS2_PLACEMENT_3D('',#223902,#129151,#129152);
#106166=AXIS2_PLACEMENT_3D('',#223905,#129153,#129154);
#106167=AXIS2_PLACEMENT_3D('',#223909,#129156,#129157);
#106168=AXIS2_PLACEMENT_3D('',#223911,#129158,#129159);
#106169=AXIS2_PLACEMENT_3D('',#223913,#129160,#129161);
#106170=AXIS2_PLACEMENT_3D('',#223915,#129163,#129164);
#106171=AXIS2_PLACEMENT_3D('',#223919,#129166,#129167);
#106172=AXIS2_PLACEMENT_3D('',#223921,#129169,#129170);
#106173=AXIS2_PLACEMENT_3D('',#223924,#129171,#129172);
#106174=AXIS2_PLACEMENT_3D('',#223928,#129174,#129175);
#106175=AXIS2_PLACEMENT_3D('',#223930,#129177,#129178);
#106176=AXIS2_PLACEMENT_3D('',#223933,#129179,#129180);
#106177=AXIS2_PLACEMENT_3D('',#223937,#129182,#129183);
#106178=AXIS2_PLACEMENT_3D('',#223939,#129184,#129185);
#106179=AXIS2_PLACEMENT_3D('',#223941,#129186,#129187);
#106180=AXIS2_PLACEMENT_3D('',#223943,#129189,#129190);
#106181=AXIS2_PLACEMENT_3D('',#223947,#129192,#129193);
#106182=AXIS2_PLACEMENT_3D('',#223949,#129195,#129196);
#106183=AXIS2_PLACEMENT_3D('',#223950,#129197,#129198);
#106184=AXIS2_PLACEMENT_3D('',#223951,#129199,#129200);
#106185=AXIS2_PLACEMENT_3D('',#223952,#129201,#129202);
#106186=AXIS2_PLACEMENT_3D('',#223953,#129203,#129204);
#106187=AXIS2_PLACEMENT_3D('',#223954,#129205,#129206);
#106188=AXIS2_PLACEMENT_3D('',#223955,#129207,#129208);
#106189=AXIS2_PLACEMENT_3D('',#223956,#129209,#129210);
#106190=AXIS2_PLACEMENT_3D('',#223957,#129211,#129212);
#106191=AXIS2_PLACEMENT_3D('',#223958,#129213,#129214);
#106192=AXIS2_PLACEMENT_3D('',#223959,#129215,#129216);
#106193=AXIS2_PLACEMENT_3D('',#223960,#129217,#129218);
#106194=AXIS2_PLACEMENT_3D('',#223961,#129219,#129220);
#106195=AXIS2_PLACEMENT_3D('',#223964,#129221,#129222);
#106196=AXIS2_PLACEMENT_3D('',#223968,#129224,#129225);
#106197=AXIS2_PLACEMENT_3D('',#223970,#129226,#129227);
#106198=AXIS2_PLACEMENT_3D('',#223972,#129228,#129229);
#106199=AXIS2_PLACEMENT_3D('',#223974,#129231,#129232);
#106200=AXIS2_PLACEMENT_3D('',#223978,#129234,#129235);
#106201=AXIS2_PLACEMENT_3D('',#223980,#129237,#129238);
#106202=AXIS2_PLACEMENT_3D('',#223983,#129239,#129240);
#106203=AXIS2_PLACEMENT_3D('',#223987,#129242,#129243);
#106204=AXIS2_PLACEMENT_3D('',#223989,#129245,#129246);
#106205=AXIS2_PLACEMENT_3D('',#223992,#129247,#129248);
#106206=AXIS2_PLACEMENT_3D('',#223996,#129250,#129251);
#106207=AXIS2_PLACEMENT_3D('',#223998,#129252,#129253);
#106208=AXIS2_PLACEMENT_3D('',#224000,#129254,#129255);
#106209=AXIS2_PLACEMENT_3D('',#224002,#129257,#129258);
#106210=AXIS2_PLACEMENT_3D('',#224006,#129260,#129261);
#106211=AXIS2_PLACEMENT_3D('',#224008,#129263,#129264);
#106212=AXIS2_PLACEMENT_3D('',#224009,#129265,#129266);
#106213=AXIS2_PLACEMENT_3D('',#224010,#129267,#129268);
#106214=AXIS2_PLACEMENT_3D('',#224011,#129269,#129270);
#106215=AXIS2_PLACEMENT_3D('',#224012,#129271,#129272);
#106216=AXIS2_PLACEMENT_3D('',#224013,#129273,#129274);
#106217=AXIS2_PLACEMENT_3D('',#224014,#129275,#129276);
#106218=AXIS2_PLACEMENT_3D('',#224015,#129277,#129278);
#106219=AXIS2_PLACEMENT_3D('',#224016,#129279,#129280);
#106220=AXIS2_PLACEMENT_3D('',#224017,#129281,#129282);
#106221=AXIS2_PLACEMENT_3D('',#224018,#129283,#129284);
#106222=AXIS2_PLACEMENT_3D('',#224019,#129285,#129286);
#106223=AXIS2_PLACEMENT_3D('',#224020,#129287,#129288);
#106224=AXIS2_PLACEMENT_3D('',#224023,#129289,#129290);
#106225=AXIS2_PLACEMENT_3D('',#224027,#129292,#129293);
#106226=AXIS2_PLACEMENT_3D('',#224029,#129294,#129295);
#106227=AXIS2_PLACEMENT_3D('',#224031,#129296,#129297);
#106228=AXIS2_PLACEMENT_3D('',#224033,#129299,#129300);
#106229=AXIS2_PLACEMENT_3D('',#224037,#129302,#129303);
#106230=AXIS2_PLACEMENT_3D('',#224039,#129305,#129306);
#106231=AXIS2_PLACEMENT_3D('',#224042,#129307,#129308);
#106232=AXIS2_PLACEMENT_3D('',#224046,#129310,#129311);
#106233=AXIS2_PLACEMENT_3D('',#224048,#129313,#129314);
#106234=AXIS2_PLACEMENT_3D('',#224051,#129315,#129316);
#106235=AXIS2_PLACEMENT_3D('',#224055,#129318,#129319);
#106236=AXIS2_PLACEMENT_3D('',#224057,#129320,#129321);
#106237=AXIS2_PLACEMENT_3D('',#224059,#129322,#129323);
#106238=AXIS2_PLACEMENT_3D('',#224061,#129325,#129326);
#106239=AXIS2_PLACEMENT_3D('',#224065,#129328,#129329);
#106240=AXIS2_PLACEMENT_3D('',#224067,#129331,#129332);
#106241=AXIS2_PLACEMENT_3D('',#224068,#129333,#129334);
#106242=AXIS2_PLACEMENT_3D('',#224069,#129335,#129336);
#106243=AXIS2_PLACEMENT_3D('',#224070,#129337,#129338);
#106244=AXIS2_PLACEMENT_3D('',#224071,#129339,#129340);
#106245=AXIS2_PLACEMENT_3D('',#224072,#129341,#129342);
#106246=AXIS2_PLACEMENT_3D('',#224073,#129343,#129344);
#106247=AXIS2_PLACEMENT_3D('',#224074,#129345,#129346);
#106248=AXIS2_PLACEMENT_3D('',#224075,#129347,#129348);
#106249=AXIS2_PLACEMENT_3D('',#224076,#129349,#129350);
#106250=AXIS2_PLACEMENT_3D('',#224077,#129351,#129352);
#106251=AXIS2_PLACEMENT_3D('',#224078,#129353,#129354);
#106252=AXIS2_PLACEMENT_3D('',#224079,#129355,#129356);
#106253=AXIS2_PLACEMENT_3D('',#224082,#129357,#129358);
#106254=AXIS2_PLACEMENT_3D('',#224086,#129360,#129361);
#106255=AXIS2_PLACEMENT_3D('',#224088,#129362,#129363);
#106256=AXIS2_PLACEMENT_3D('',#224090,#129364,#129365);
#106257=AXIS2_PLACEMENT_3D('',#224092,#129367,#129368);
#106258=AXIS2_PLACEMENT_3D('',#224096,#129370,#129371);
#106259=AXIS2_PLACEMENT_3D('',#224098,#129373,#129374);
#106260=AXIS2_PLACEMENT_3D('',#224101,#129375,#129376);
#106261=AXIS2_PLACEMENT_3D('',#224105,#129378,#129379);
#106262=AXIS2_PLACEMENT_3D('',#224107,#129381,#129382);
#106263=AXIS2_PLACEMENT_3D('',#224110,#129383,#129384);
#106264=AXIS2_PLACEMENT_3D('',#224114,#129386,#129387);
#106265=AXIS2_PLACEMENT_3D('',#224116,#129388,#129389);
#106266=AXIS2_PLACEMENT_3D('',#224118,#129390,#129391);
#106267=AXIS2_PLACEMENT_3D('',#224120,#129393,#129394);
#106268=AXIS2_PLACEMENT_3D('',#224124,#129396,#129397);
#106269=AXIS2_PLACEMENT_3D('',#224126,#129399,#129400);
#106270=AXIS2_PLACEMENT_3D('',#224127,#129401,#129402);
#106271=AXIS2_PLACEMENT_3D('',#224128,#129403,#129404);
#106272=AXIS2_PLACEMENT_3D('',#224129,#129405,#129406);
#106273=AXIS2_PLACEMENT_3D('',#224130,#129407,#129408);
#106274=AXIS2_PLACEMENT_3D('',#224131,#129409,#129410);
#106275=AXIS2_PLACEMENT_3D('',#224132,#129411,#129412);
#106276=AXIS2_PLACEMENT_3D('',#224133,#129413,#129414);
#106277=AXIS2_PLACEMENT_3D('',#224134,#129415,#129416);
#106278=AXIS2_PLACEMENT_3D('',#224135,#129417,#129418);
#106279=AXIS2_PLACEMENT_3D('',#224136,#129419,#129420);
#106280=AXIS2_PLACEMENT_3D('',#224137,#129421,#129422);
#106281=AXIS2_PLACEMENT_3D('',#224138,#129423,#129424);
#106282=AXIS2_PLACEMENT_3D('',#224141,#129425,#129426);
#106283=AXIS2_PLACEMENT_3D('',#224145,#129428,#129429);
#106284=AXIS2_PLACEMENT_3D('',#224147,#129430,#129431);
#106285=AXIS2_PLACEMENT_3D('',#224149,#129432,#129433);
#106286=AXIS2_PLACEMENT_3D('',#224151,#129435,#129436);
#106287=AXIS2_PLACEMENT_3D('',#224155,#129438,#129439);
#106288=AXIS2_PLACEMENT_3D('',#224157,#129441,#129442);
#106289=AXIS2_PLACEMENT_3D('',#224160,#129443,#129444);
#106290=AXIS2_PLACEMENT_3D('',#224164,#129446,#129447);
#106291=AXIS2_PLACEMENT_3D('',#224166,#129449,#129450);
#106292=AXIS2_PLACEMENT_3D('',#224169,#129451,#129452);
#106293=AXIS2_PLACEMENT_3D('',#224173,#129454,#129455);
#106294=AXIS2_PLACEMENT_3D('',#224175,#129456,#129457);
#106295=AXIS2_PLACEMENT_3D('',#224177,#129458,#129459);
#106296=AXIS2_PLACEMENT_3D('',#224179,#129461,#129462);
#106297=AXIS2_PLACEMENT_3D('',#224183,#129464,#129465);
#106298=AXIS2_PLACEMENT_3D('',#224185,#129467,#129468);
#106299=AXIS2_PLACEMENT_3D('',#224186,#129469,#129470);
#106300=AXIS2_PLACEMENT_3D('',#224187,#129471,#129472);
#106301=AXIS2_PLACEMENT_3D('',#224188,#129473,#129474);
#106302=AXIS2_PLACEMENT_3D('',#224189,#129475,#129476);
#106303=AXIS2_PLACEMENT_3D('',#224190,#129477,#129478);
#106304=AXIS2_PLACEMENT_3D('',#224191,#129479,#129480);
#106305=AXIS2_PLACEMENT_3D('',#224192,#129481,#129482);
#106306=AXIS2_PLACEMENT_3D('',#224193,#129483,#129484);
#106307=AXIS2_PLACEMENT_3D('',#224194,#129485,#129486);
#106308=AXIS2_PLACEMENT_3D('',#224195,#129487,#129488);
#106309=AXIS2_PLACEMENT_3D('',#224196,#129489,#129490);
#106310=AXIS2_PLACEMENT_3D('',#224197,#129491,#129492);
#106311=AXIS2_PLACEMENT_3D('',#224200,#129493,#129494);
#106312=AXIS2_PLACEMENT_3D('',#224204,#129496,#129497);
#106313=AXIS2_PLACEMENT_3D('',#224206,#129498,#129499);
#106314=AXIS2_PLACEMENT_3D('',#224208,#129500,#129501);
#106315=AXIS2_PLACEMENT_3D('',#224210,#129503,#129504);
#106316=AXIS2_PLACEMENT_3D('',#224214,#129506,#129507);
#106317=AXIS2_PLACEMENT_3D('',#224216,#129509,#129510);
#106318=AXIS2_PLACEMENT_3D('',#224219,#129511,#129512);
#106319=AXIS2_PLACEMENT_3D('',#224223,#129514,#129515);
#106320=AXIS2_PLACEMENT_3D('',#224225,#129517,#129518);
#106321=AXIS2_PLACEMENT_3D('',#224228,#129519,#129520);
#106322=AXIS2_PLACEMENT_3D('',#224232,#129522,#129523);
#106323=AXIS2_PLACEMENT_3D('',#224234,#129524,#129525);
#106324=AXIS2_PLACEMENT_3D('',#224236,#129526,#129527);
#106325=AXIS2_PLACEMENT_3D('',#224238,#129529,#129530);
#106326=AXIS2_PLACEMENT_3D('',#224242,#129532,#129533);
#106327=AXIS2_PLACEMENT_3D('',#224244,#129535,#129536);
#106328=AXIS2_PLACEMENT_3D('',#224245,#129537,#129538);
#106329=AXIS2_PLACEMENT_3D('',#224246,#129539,#129540);
#106330=AXIS2_PLACEMENT_3D('',#224247,#129541,#129542);
#106331=AXIS2_PLACEMENT_3D('',#224248,#129543,#129544);
#106332=AXIS2_PLACEMENT_3D('',#224249,#129545,#129546);
#106333=AXIS2_PLACEMENT_3D('',#224250,#129547,#129548);
#106334=AXIS2_PLACEMENT_3D('',#224251,#129549,#129550);
#106335=AXIS2_PLACEMENT_3D('',#224252,#129551,#129552);
#106336=AXIS2_PLACEMENT_3D('',#224253,#129553,#129554);
#106337=AXIS2_PLACEMENT_3D('',#224254,#129555,#129556);
#106338=AXIS2_PLACEMENT_3D('',#224255,#129557,#129558);
#106339=AXIS2_PLACEMENT_3D('',#224256,#129559,#129560);
#106340=AXIS2_PLACEMENT_3D('',#224259,#129561,#129562);
#106341=AXIS2_PLACEMENT_3D('',#224263,#129564,#129565);
#106342=AXIS2_PLACEMENT_3D('',#224265,#129566,#129567);
#106343=AXIS2_PLACEMENT_3D('',#224267,#129568,#129569);
#106344=AXIS2_PLACEMENT_3D('',#224269,#129571,#129572);
#106345=AXIS2_PLACEMENT_3D('',#224273,#129574,#129575);
#106346=AXIS2_PLACEMENT_3D('',#224275,#129577,#129578);
#106347=AXIS2_PLACEMENT_3D('',#224278,#129579,#129580);
#106348=AXIS2_PLACEMENT_3D('',#224282,#129582,#129583);
#106349=AXIS2_PLACEMENT_3D('',#224284,#129585,#129586);
#106350=AXIS2_PLACEMENT_3D('',#224287,#129587,#129588);
#106351=AXIS2_PLACEMENT_3D('',#224291,#129590,#129591);
#106352=AXIS2_PLACEMENT_3D('',#224293,#129592,#129593);
#106353=AXIS2_PLACEMENT_3D('',#224295,#129594,#129595);
#106354=AXIS2_PLACEMENT_3D('',#224297,#129597,#129598);
#106355=AXIS2_PLACEMENT_3D('',#224301,#129600,#129601);
#106356=AXIS2_PLACEMENT_3D('',#224303,#129603,#129604);
#106357=AXIS2_PLACEMENT_3D('',#224304,#129605,#129606);
#106358=AXIS2_PLACEMENT_3D('',#224305,#129607,#129608);
#106359=AXIS2_PLACEMENT_3D('',#224306,#129609,#129610);
#106360=AXIS2_PLACEMENT_3D('',#224307,#129611,#129612);
#106361=AXIS2_PLACEMENT_3D('',#224308,#129613,#129614);
#106362=AXIS2_PLACEMENT_3D('',#224309,#129615,#129616);
#106363=AXIS2_PLACEMENT_3D('',#224310,#129617,#129618);
#106364=AXIS2_PLACEMENT_3D('',#224311,#129619,#129620);
#106365=AXIS2_PLACEMENT_3D('',#224312,#129621,#129622);
#106366=AXIS2_PLACEMENT_3D('',#224313,#129623,#129624);
#106367=AXIS2_PLACEMENT_3D('',#224314,#129625,#129626);
#106368=AXIS2_PLACEMENT_3D('',#224315,#129627,#129628);
#106369=AXIS2_PLACEMENT_3D('',#224318,#129629,#129630);
#106370=AXIS2_PLACEMENT_3D('',#224322,#129632,#129633);
#106371=AXIS2_PLACEMENT_3D('',#224324,#129634,#129635);
#106372=AXIS2_PLACEMENT_3D('',#224326,#129636,#129637);
#106373=AXIS2_PLACEMENT_3D('',#224328,#129639,#129640);
#106374=AXIS2_PLACEMENT_3D('',#224332,#129642,#129643);
#106375=AXIS2_PLACEMENT_3D('',#224334,#129645,#129646);
#106376=AXIS2_PLACEMENT_3D('',#224337,#129647,#129648);
#106377=AXIS2_PLACEMENT_3D('',#224341,#129650,#129651);
#106378=AXIS2_PLACEMENT_3D('',#224343,#129653,#129654);
#106379=AXIS2_PLACEMENT_3D('',#224346,#129655,#129656);
#106380=AXIS2_PLACEMENT_3D('',#224350,#129658,#129659);
#106381=AXIS2_PLACEMENT_3D('',#224352,#129660,#129661);
#106382=AXIS2_PLACEMENT_3D('',#224354,#129662,#129663);
#106383=AXIS2_PLACEMENT_3D('',#224356,#129665,#129666);
#106384=AXIS2_PLACEMENT_3D('',#224360,#129668,#129669);
#106385=AXIS2_PLACEMENT_3D('',#224362,#129671,#129672);
#106386=AXIS2_PLACEMENT_3D('',#224363,#129673,#129674);
#106387=AXIS2_PLACEMENT_3D('',#224364,#129675,#129676);
#106388=AXIS2_PLACEMENT_3D('',#224365,#129677,#129678);
#106389=AXIS2_PLACEMENT_3D('',#224366,#129679,#129680);
#106390=AXIS2_PLACEMENT_3D('',#224367,#129681,#129682);
#106391=AXIS2_PLACEMENT_3D('',#224368,#129683,#129684);
#106392=AXIS2_PLACEMENT_3D('',#224369,#129685,#129686);
#106393=AXIS2_PLACEMENT_3D('',#224370,#129687,#129688);
#106394=AXIS2_PLACEMENT_3D('',#224371,#129689,#129690);
#106395=AXIS2_PLACEMENT_3D('',#224372,#129691,#129692);
#106396=AXIS2_PLACEMENT_3D('',#224373,#129693,#129694);
#106397=AXIS2_PLACEMENT_3D('',#224374,#129695,#129696);
#106398=AXIS2_PLACEMENT_3D('',#224377,#129697,#129698);
#106399=AXIS2_PLACEMENT_3D('',#224381,#129700,#129701);
#106400=AXIS2_PLACEMENT_3D('',#224383,#129702,#129703);
#106401=AXIS2_PLACEMENT_3D('',#224385,#129704,#129705);
#106402=AXIS2_PLACEMENT_3D('',#224387,#129707,#129708);
#106403=AXIS2_PLACEMENT_3D('',#224391,#129710,#129711);
#106404=AXIS2_PLACEMENT_3D('',#224393,#129713,#129714);
#106405=AXIS2_PLACEMENT_3D('',#224396,#129715,#129716);
#106406=AXIS2_PLACEMENT_3D('',#224400,#129718,#129719);
#106407=AXIS2_PLACEMENT_3D('',#224402,#129721,#129722);
#106408=AXIS2_PLACEMENT_3D('',#224405,#129723,#129724);
#106409=AXIS2_PLACEMENT_3D('',#224409,#129726,#129727);
#106410=AXIS2_PLACEMENT_3D('',#224411,#129728,#129729);
#106411=AXIS2_PLACEMENT_3D('',#224413,#129730,#129731);
#106412=AXIS2_PLACEMENT_3D('',#224415,#129733,#129734);
#106413=AXIS2_PLACEMENT_3D('',#224419,#129736,#129737);
#106414=AXIS2_PLACEMENT_3D('',#224421,#129739,#129740);
#106415=AXIS2_PLACEMENT_3D('',#224422,#129741,#129742);
#106416=AXIS2_PLACEMENT_3D('',#224423,#129743,#129744);
#106417=AXIS2_PLACEMENT_3D('',#224424,#129745,#129746);
#106418=AXIS2_PLACEMENT_3D('',#224425,#129747,#129748);
#106419=AXIS2_PLACEMENT_3D('',#224426,#129749,#129750);
#106420=AXIS2_PLACEMENT_3D('',#224427,#129751,#129752);
#106421=AXIS2_PLACEMENT_3D('',#224428,#129753,#129754);
#106422=AXIS2_PLACEMENT_3D('',#224429,#129755,#129756);
#106423=AXIS2_PLACEMENT_3D('',#224430,#129757,#129758);
#106424=AXIS2_PLACEMENT_3D('',#224431,#129759,#129760);
#106425=AXIS2_PLACEMENT_3D('',#224432,#129761,#129762);
#106426=AXIS2_PLACEMENT_3D('',#224433,#129763,#129764);
#106427=AXIS2_PLACEMENT_3D('',#224436,#129765,#129766);
#106428=AXIS2_PLACEMENT_3D('',#224440,#129768,#129769);
#106429=AXIS2_PLACEMENT_3D('',#224442,#129770,#129771);
#106430=AXIS2_PLACEMENT_3D('',#224444,#129772,#129773);
#106431=AXIS2_PLACEMENT_3D('',#224446,#129775,#129776);
#106432=AXIS2_PLACEMENT_3D('',#224450,#129778,#129779);
#106433=AXIS2_PLACEMENT_3D('',#224452,#129781,#129782);
#106434=AXIS2_PLACEMENT_3D('',#224455,#129783,#129784);
#106435=AXIS2_PLACEMENT_3D('',#224459,#129786,#129787);
#106436=AXIS2_PLACEMENT_3D('',#224461,#129789,#129790);
#106437=AXIS2_PLACEMENT_3D('',#224464,#129791,#129792);
#106438=AXIS2_PLACEMENT_3D('',#224468,#129794,#129795);
#106439=AXIS2_PLACEMENT_3D('',#224470,#129796,#129797);
#106440=AXIS2_PLACEMENT_3D('',#224472,#129798,#129799);
#106441=AXIS2_PLACEMENT_3D('',#224474,#129801,#129802);
#106442=AXIS2_PLACEMENT_3D('',#224478,#129804,#129805);
#106443=AXIS2_PLACEMENT_3D('',#224480,#129807,#129808);
#106444=AXIS2_PLACEMENT_3D('',#224481,#129809,#129810);
#106445=AXIS2_PLACEMENT_3D('',#224482,#129811,#129812);
#106446=AXIS2_PLACEMENT_3D('',#224483,#129813,#129814);
#106447=AXIS2_PLACEMENT_3D('',#224484,#129815,#129816);
#106448=AXIS2_PLACEMENT_3D('',#224485,#129817,#129818);
#106449=AXIS2_PLACEMENT_3D('',#224486,#129819,#129820);
#106450=AXIS2_PLACEMENT_3D('',#224487,#129821,#129822);
#106451=AXIS2_PLACEMENT_3D('',#224488,#129823,#129824);
#106452=AXIS2_PLACEMENT_3D('',#224489,#129825,#129826);
#106453=AXIS2_PLACEMENT_3D('',#224490,#129827,#129828);
#106454=AXIS2_PLACEMENT_3D('',#224491,#129829,#129830);
#106455=AXIS2_PLACEMENT_3D('',#224492,#129831,#129832);
#106456=AXIS2_PLACEMENT_3D('',#224495,#129833,#129834);
#106457=AXIS2_PLACEMENT_3D('',#224499,#129836,#129837);
#106458=AXIS2_PLACEMENT_3D('',#224501,#129838,#129839);
#106459=AXIS2_PLACEMENT_3D('',#224503,#129840,#129841);
#106460=AXIS2_PLACEMENT_3D('',#224505,#129843,#129844);
#106461=AXIS2_PLACEMENT_3D('',#224509,#129846,#129847);
#106462=AXIS2_PLACEMENT_3D('',#224511,#129849,#129850);
#106463=AXIS2_PLACEMENT_3D('',#224514,#129851,#129852);
#106464=AXIS2_PLACEMENT_3D('',#224518,#129854,#129855);
#106465=AXIS2_PLACEMENT_3D('',#224520,#129857,#129858);
#106466=AXIS2_PLACEMENT_3D('',#224523,#129859,#129860);
#106467=AXIS2_PLACEMENT_3D('',#224527,#129862,#129863);
#106468=AXIS2_PLACEMENT_3D('',#224529,#129864,#129865);
#106469=AXIS2_PLACEMENT_3D('',#224531,#129866,#129867);
#106470=AXIS2_PLACEMENT_3D('',#224533,#129869,#129870);
#106471=AXIS2_PLACEMENT_3D('',#224537,#129872,#129873);
#106472=AXIS2_PLACEMENT_3D('',#224539,#129875,#129876);
#106473=AXIS2_PLACEMENT_3D('',#224540,#129877,#129878);
#106474=AXIS2_PLACEMENT_3D('',#224541,#129879,#129880);
#106475=AXIS2_PLACEMENT_3D('',#224542,#129881,#129882);
#106476=AXIS2_PLACEMENT_3D('',#224543,#129883,#129884);
#106477=AXIS2_PLACEMENT_3D('',#224544,#129885,#129886);
#106478=AXIS2_PLACEMENT_3D('',#224545,#129887,#129888);
#106479=AXIS2_PLACEMENT_3D('',#224546,#129889,#129890);
#106480=AXIS2_PLACEMENT_3D('',#224547,#129891,#129892);
#106481=AXIS2_PLACEMENT_3D('',#224548,#129893,#129894);
#106482=AXIS2_PLACEMENT_3D('',#224549,#129895,#129896);
#106483=AXIS2_PLACEMENT_3D('',#224550,#129897,#129898);
#106484=AXIS2_PLACEMENT_3D('',#224551,#129899,#129900);
#106485=AXIS2_PLACEMENT_3D('',#224554,#129901,#129902);
#106486=AXIS2_PLACEMENT_3D('',#224558,#129904,#129905);
#106487=AXIS2_PLACEMENT_3D('',#224560,#129906,#129907);
#106488=AXIS2_PLACEMENT_3D('',#224562,#129908,#129909);
#106489=AXIS2_PLACEMENT_3D('',#224564,#129911,#129912);
#106490=AXIS2_PLACEMENT_3D('',#224568,#129914,#129915);
#106491=AXIS2_PLACEMENT_3D('',#224570,#129917,#129918);
#106492=AXIS2_PLACEMENT_3D('',#224573,#129919,#129920);
#106493=AXIS2_PLACEMENT_3D('',#224577,#129922,#129923);
#106494=AXIS2_PLACEMENT_3D('',#224579,#129925,#129926);
#106495=AXIS2_PLACEMENT_3D('',#224582,#129927,#129928);
#106496=AXIS2_PLACEMENT_3D('',#224586,#129930,#129931);
#106497=AXIS2_PLACEMENT_3D('',#224588,#129932,#129933);
#106498=AXIS2_PLACEMENT_3D('',#224590,#129934,#129935);
#106499=AXIS2_PLACEMENT_3D('',#224592,#129937,#129938);
#106500=AXIS2_PLACEMENT_3D('',#224596,#129940,#129941);
#106501=AXIS2_PLACEMENT_3D('',#224598,#129943,#129944);
#106502=AXIS2_PLACEMENT_3D('',#224599,#129945,#129946);
#106503=AXIS2_PLACEMENT_3D('',#224600,#129947,#129948);
#106504=AXIS2_PLACEMENT_3D('',#224601,#129949,#129950);
#106505=AXIS2_PLACEMENT_3D('',#224602,#129951,#129952);
#106506=AXIS2_PLACEMENT_3D('',#224603,#129953,#129954);
#106507=AXIS2_PLACEMENT_3D('',#224604,#129955,#129956);
#106508=AXIS2_PLACEMENT_3D('',#224605,#129957,#129958);
#106509=AXIS2_PLACEMENT_3D('',#224606,#129959,#129960);
#106510=AXIS2_PLACEMENT_3D('',#224607,#129961,#129962);
#106511=AXIS2_PLACEMENT_3D('',#224608,#129963,#129964);
#106512=AXIS2_PLACEMENT_3D('',#224609,#129965,#129966);
#106513=AXIS2_PLACEMENT_3D('',#224610,#129967,#129968);
#106514=AXIS2_PLACEMENT_3D('',#224613,#129969,#129970);
#106515=AXIS2_PLACEMENT_3D('',#224617,#129972,#129973);
#106516=AXIS2_PLACEMENT_3D('',#224619,#129974,#129975);
#106517=AXIS2_PLACEMENT_3D('',#224621,#129976,#129977);
#106518=AXIS2_PLACEMENT_3D('',#224623,#129979,#129980);
#106519=AXIS2_PLACEMENT_3D('',#224627,#129982,#129983);
#106520=AXIS2_PLACEMENT_3D('',#224629,#129985,#129986);
#106521=AXIS2_PLACEMENT_3D('',#224632,#129987,#129988);
#106522=AXIS2_PLACEMENT_3D('',#224636,#129990,#129991);
#106523=AXIS2_PLACEMENT_3D('',#224638,#129993,#129994);
#106524=AXIS2_PLACEMENT_3D('',#224641,#129995,#129996);
#106525=AXIS2_PLACEMENT_3D('',#224645,#129998,#129999);
#106526=AXIS2_PLACEMENT_3D('',#224647,#130000,#130001);
#106527=AXIS2_PLACEMENT_3D('',#224649,#130002,#130003);
#106528=AXIS2_PLACEMENT_3D('',#224651,#130005,#130006);
#106529=AXIS2_PLACEMENT_3D('',#224655,#130008,#130009);
#106530=AXIS2_PLACEMENT_3D('',#224657,#130011,#130012);
#106531=AXIS2_PLACEMENT_3D('',#224658,#130013,#130014);
#106532=AXIS2_PLACEMENT_3D('',#224659,#130015,#130016);
#106533=AXIS2_PLACEMENT_3D('',#224660,#130017,#130018);
#106534=AXIS2_PLACEMENT_3D('',#224661,#130019,#130020);
#106535=AXIS2_PLACEMENT_3D('',#224662,#130021,#130022);
#106536=AXIS2_PLACEMENT_3D('',#224663,#130023,#130024);
#106537=AXIS2_PLACEMENT_3D('',#224664,#130025,#130026);
#106538=AXIS2_PLACEMENT_3D('',#224665,#130027,#130028);
#106539=AXIS2_PLACEMENT_3D('',#224666,#130029,#130030);
#106540=AXIS2_PLACEMENT_3D('',#224667,#130031,#130032);
#106541=AXIS2_PLACEMENT_3D('',#224668,#130033,#130034);
#106542=AXIS2_PLACEMENT_3D('',#224669,#130035,#130036);
#106543=AXIS2_PLACEMENT_3D('',#224672,#130037,#130038);
#106544=AXIS2_PLACEMENT_3D('',#224676,#130040,#130041);
#106545=AXIS2_PLACEMENT_3D('',#224678,#130042,#130043);
#106546=AXIS2_PLACEMENT_3D('',#224680,#130044,#130045);
#106547=AXIS2_PLACEMENT_3D('',#224682,#130047,#130048);
#106548=AXIS2_PLACEMENT_3D('',#224686,#130050,#130051);
#106549=AXIS2_PLACEMENT_3D('',#224688,#130053,#130054);
#106550=AXIS2_PLACEMENT_3D('',#224691,#130055,#130056);
#106551=AXIS2_PLACEMENT_3D('',#224695,#130058,#130059);
#106552=AXIS2_PLACEMENT_3D('',#224697,#130061,#130062);
#106553=AXIS2_PLACEMENT_3D('',#224700,#130063,#130064);
#106554=AXIS2_PLACEMENT_3D('',#224704,#130066,#130067);
#106555=AXIS2_PLACEMENT_3D('',#224706,#130068,#130069);
#106556=AXIS2_PLACEMENT_3D('',#224708,#130070,#130071);
#106557=AXIS2_PLACEMENT_3D('',#224710,#130073,#130074);
#106558=AXIS2_PLACEMENT_3D('',#224714,#130076,#130077);
#106559=AXIS2_PLACEMENT_3D('',#224716,#130079,#130080);
#106560=AXIS2_PLACEMENT_3D('',#224717,#130081,#130082);
#106561=AXIS2_PLACEMENT_3D('',#224718,#130083,#130084);
#106562=AXIS2_PLACEMENT_3D('',#224719,#130085,#130086);
#106563=AXIS2_PLACEMENT_3D('',#224720,#130087,#130088);
#106564=AXIS2_PLACEMENT_3D('',#224721,#130089,#130090);
#106565=AXIS2_PLACEMENT_3D('',#224722,#130091,#130092);
#106566=AXIS2_PLACEMENT_3D('',#224723,#130093,#130094);
#106567=AXIS2_PLACEMENT_3D('',#224724,#130095,#130096);
#106568=AXIS2_PLACEMENT_3D('',#224725,#130097,#130098);
#106569=AXIS2_PLACEMENT_3D('',#224726,#130099,#130100);
#106570=AXIS2_PLACEMENT_3D('',#224727,#130101,#130102);
#106571=AXIS2_PLACEMENT_3D('',#224728,#130103,#130104);
#106572=AXIS2_PLACEMENT_3D('',#224731,#130105,#130106);
#106573=AXIS2_PLACEMENT_3D('',#224735,#130108,#130109);
#106574=AXIS2_PLACEMENT_3D('',#224737,#130110,#130111);
#106575=AXIS2_PLACEMENT_3D('',#224739,#130112,#130113);
#106576=AXIS2_PLACEMENT_3D('',#224741,#130115,#130116);
#106577=AXIS2_PLACEMENT_3D('',#224745,#130118,#130119);
#106578=AXIS2_PLACEMENT_3D('',#224747,#130121,#130122);
#106579=AXIS2_PLACEMENT_3D('',#224750,#130123,#130124);
#106580=AXIS2_PLACEMENT_3D('',#224754,#130126,#130127);
#106581=AXIS2_PLACEMENT_3D('',#224756,#130129,#130130);
#106582=AXIS2_PLACEMENT_3D('',#224759,#130131,#130132);
#106583=AXIS2_PLACEMENT_3D('',#224763,#130134,#130135);
#106584=AXIS2_PLACEMENT_3D('',#224765,#130136,#130137);
#106585=AXIS2_PLACEMENT_3D('',#224767,#130138,#130139);
#106586=AXIS2_PLACEMENT_3D('',#224769,#130141,#130142);
#106587=AXIS2_PLACEMENT_3D('',#224773,#130144,#130145);
#106588=AXIS2_PLACEMENT_3D('',#224775,#130147,#130148);
#106589=AXIS2_PLACEMENT_3D('',#224776,#130149,#130150);
#106590=AXIS2_PLACEMENT_3D('',#224777,#130151,#130152);
#106591=AXIS2_PLACEMENT_3D('',#224778,#130153,#130154);
#106592=AXIS2_PLACEMENT_3D('',#224779,#130155,#130156);
#106593=AXIS2_PLACEMENT_3D('',#224780,#130157,#130158);
#106594=AXIS2_PLACEMENT_3D('',#224781,#130159,#130160);
#106595=AXIS2_PLACEMENT_3D('',#224782,#130161,#130162);
#106596=AXIS2_PLACEMENT_3D('',#224783,#130163,#130164);
#106597=AXIS2_PLACEMENT_3D('',#224784,#130165,#130166);
#106598=AXIS2_PLACEMENT_3D('',#224785,#130167,#130168);
#106599=AXIS2_PLACEMENT_3D('',#224786,#130169,#130170);
#106600=AXIS2_PLACEMENT_3D('',#224787,#130171,#130172);
#106601=AXIS2_PLACEMENT_3D('',#224790,#130173,#130174);
#106602=AXIS2_PLACEMENT_3D('',#224794,#130176,#130177);
#106603=AXIS2_PLACEMENT_3D('',#224796,#130178,#130179);
#106604=AXIS2_PLACEMENT_3D('',#224798,#130180,#130181);
#106605=AXIS2_PLACEMENT_3D('',#224800,#130183,#130184);
#106606=AXIS2_PLACEMENT_3D('',#224804,#130186,#130187);
#106607=AXIS2_PLACEMENT_3D('',#224806,#130189,#130190);
#106608=AXIS2_PLACEMENT_3D('',#224809,#130191,#130192);
#106609=AXIS2_PLACEMENT_3D('',#224813,#130194,#130195);
#106610=AXIS2_PLACEMENT_3D('',#224815,#130197,#130198);
#106611=AXIS2_PLACEMENT_3D('',#224818,#130199,#130200);
#106612=AXIS2_PLACEMENT_3D('',#224822,#130202,#130203);
#106613=AXIS2_PLACEMENT_3D('',#224824,#130204,#130205);
#106614=AXIS2_PLACEMENT_3D('',#224826,#130206,#130207);
#106615=AXIS2_PLACEMENT_3D('',#224828,#130209,#130210);
#106616=AXIS2_PLACEMENT_3D('',#224832,#130212,#130213);
#106617=AXIS2_PLACEMENT_3D('',#224834,#130215,#130216);
#106618=AXIS2_PLACEMENT_3D('',#224835,#130217,#130218);
#106619=AXIS2_PLACEMENT_3D('',#224836,#130219,#130220);
#106620=AXIS2_PLACEMENT_3D('',#224837,#130221,#130222);
#106621=AXIS2_PLACEMENT_3D('',#224838,#130223,#130224);
#106622=AXIS2_PLACEMENT_3D('',#224839,#130225,#130226);
#106623=AXIS2_PLACEMENT_3D('',#224840,#130227,#130228);
#106624=AXIS2_PLACEMENT_3D('',#224841,#130229,#130230);
#106625=AXIS2_PLACEMENT_3D('',#224842,#130231,#130232);
#106626=AXIS2_PLACEMENT_3D('',#224843,#130233,#130234);
#106627=AXIS2_PLACEMENT_3D('',#224844,#130235,#130236);
#106628=AXIS2_PLACEMENT_3D('',#224845,#130237,#130238);
#106629=AXIS2_PLACEMENT_3D('',#224846,#130239,#130240);
#106630=AXIS2_PLACEMENT_3D('',#224847,#130241,#130242);
#106631=AXIS2_PLACEMENT_3D('',#224850,#130243,#130244);
#106632=AXIS2_PLACEMENT_3D('',#224854,#130246,#130247);
#106633=AXIS2_PLACEMENT_3D('',#224856,#130248,#130249);
#106634=AXIS2_PLACEMENT_3D('',#224858,#130250,#130251);
#106635=AXIS2_PLACEMENT_3D('',#224860,#130253,#130254);
#106636=AXIS2_PLACEMENT_3D('',#224864,#130256,#130257);
#106637=AXIS2_PLACEMENT_3D('',#224866,#130259,#130260);
#106638=AXIS2_PLACEMENT_3D('',#224869,#130261,#130262);
#106639=AXIS2_PLACEMENT_3D('',#224873,#130264,#130265);
#106640=AXIS2_PLACEMENT_3D('',#224875,#130267,#130268);
#106641=AXIS2_PLACEMENT_3D('',#224878,#130269,#130270);
#106642=AXIS2_PLACEMENT_3D('',#224882,#130272,#130273);
#106643=AXIS2_PLACEMENT_3D('',#224884,#130274,#130275);
#106644=AXIS2_PLACEMENT_3D('',#224886,#130276,#130277);
#106645=AXIS2_PLACEMENT_3D('',#224888,#130279,#130280);
#106646=AXIS2_PLACEMENT_3D('',#224892,#130282,#130283);
#106647=AXIS2_PLACEMENT_3D('',#224894,#130285,#130286);
#106648=AXIS2_PLACEMENT_3D('',#224895,#130287,#130288);
#106649=AXIS2_PLACEMENT_3D('',#224896,#130289,#130290);
#106650=AXIS2_PLACEMENT_3D('',#224897,#130291,#130292);
#106651=AXIS2_PLACEMENT_3D('',#224898,#130293,#130294);
#106652=AXIS2_PLACEMENT_3D('',#224899,#130295,#130296);
#106653=AXIS2_PLACEMENT_3D('',#224900,#130297,#130298);
#106654=AXIS2_PLACEMENT_3D('',#224901,#130299,#130300);
#106655=AXIS2_PLACEMENT_3D('',#224902,#130301,#130302);
#106656=AXIS2_PLACEMENT_3D('',#224903,#130303,#130304);
#106657=AXIS2_PLACEMENT_3D('',#224904,#130305,#130306);
#106658=AXIS2_PLACEMENT_3D('',#224905,#130307,#130308);
#106659=AXIS2_PLACEMENT_3D('',#224906,#130309,#130310);
#106660=AXIS2_PLACEMENT_3D('',#224907,#130311,#130312);
#106661=AXIS2_PLACEMENT_3D('',#224908,#130313,#130314);
#106662=AXIS2_PLACEMENT_3D('',#224913,#130316,#130317);
#106663=AXIS2_PLACEMENT_3D('',#224916,#130319,#130320);
#106664=AXIS2_PLACEMENT_3D('',#224917,#130321,#130322);
#106665=AXIS2_PLACEMENT_3D('',#224920,#130323,#130324);
#106666=AXIS2_PLACEMENT_3D('',#224928,#130328,#130329);
#106667=AXIS2_PLACEMENT_3D('',#224934,#130332,#130333);
#106668=AXIS2_PLACEMENT_3D('',#224938,#130335,#130336);
#106669=AXIS2_PLACEMENT_3D('',#224942,#130339,#130340);
#106670=AXIS2_PLACEMENT_3D('',#224945,#130341,#130342);
#106671=AXIS2_PLACEMENT_3D('',#224953,#130346,#130347);
#106672=AXIS2_PLACEMENT_3D('',#224959,#130350,#130351);
#106673=AXIS2_PLACEMENT_3D('',#224963,#130353,#130354);
#106674=AXIS2_PLACEMENT_3D('',#224967,#130357,#130358);
#106675=AXIS2_PLACEMENT_3D('',#225072,#130359,#130360);
#106676=AXIS2_PLACEMENT_3D('',#225171,#130361,#130362);
#106677=AXIS2_PLACEMENT_3D('',#225172,#130363,#130364);
#106678=AXIS2_PLACEMENT_3D('',#225173,#130365,#130366);
#106679=AXIS2_PLACEMENT_3D('',#225186,#130367,#130368);
#106680=AXIS2_PLACEMENT_3D('',#225187,#130369,#130370);
#106681=AXIS2_PLACEMENT_3D('',#225188,#130371,#130372);
#106682=AXIS2_PLACEMENT_3D('',#225189,#130373,#130374);
#106683=AXIS2_PLACEMENT_3D('',#225190,#130375,#130376);
#106684=AXIS2_PLACEMENT_3D('',#225203,#130377,#130378);
#106685=AXIS2_PLACEMENT_3D('',#225216,#130379,#130380);
#106686=AXIS2_PLACEMENT_3D('',#225217,#130381,#130382);
#106687=AXIS2_PLACEMENT_3D('',#225218,#130383,#130384);
#106688=AXIS2_PLACEMENT_3D('',#225219,#130385,#130386);
#106689=AXIS2_PLACEMENT_3D('',#225220,#130387,#130388);
#106690=AXIS2_PLACEMENT_3D('',#225239,#130389,#130390);
#106691=AXIS2_PLACEMENT_3D('',#225240,#130391,#130392);
#106692=AXIS2_PLACEMENT_3D('',#225241,#130393,#130394);
#106693=AXIS2_PLACEMENT_3D('',#225242,#130395,#130396);
#106694=AXIS2_PLACEMENT_3D('',#225243,#130397,#130398);
#106695=AXIS2_PLACEMENT_3D('',#225256,#130399,#130400);
#106696=AXIS2_PLACEMENT_3D('',#225275,#130401,#130402);
#106697=AXIS2_PLACEMENT_3D('',#225276,#130403,#130404);
#106698=AXIS2_PLACEMENT_3D('',#225277,#130405,#130406);
#106699=AXIS2_PLACEMENT_3D('',#225278,#130407,#130408);
#106700=AXIS2_PLACEMENT_3D('',#225279,#130409,#130410);
#106701=AXIS2_PLACEMENT_3D('',#225298,#130411,#130412);
#106702=AXIS2_PLACEMENT_3D('',#225311,#130413,#130414);
#106703=AXIS2_PLACEMENT_3D('',#225312,#130415,#130416);
#106704=AXIS2_PLACEMENT_3D('',#225313,#130417,#130418);
#106705=AXIS2_PLACEMENT_3D('',#225314,#130419,#130420);
#106706=AXIS2_PLACEMENT_3D('',#225315,#130421,#130422);
#106707=AXIS2_PLACEMENT_3D('',#225334,#130423,#130424);
#106708=AXIS2_PLACEMENT_3D('',#225335,#130425,#130426);
#106709=AXIS2_PLACEMENT_3D('',#225336,#130427,#130428);
#106710=AXIS2_PLACEMENT_3D('',#225337,#130429,#130430);
#106711=AXIS2_PLACEMENT_3D('',#225338,#130431,#130432);
#106712=AXIS2_PLACEMENT_3D('',#225351,#130433,#130434);
#106713=AXIS2_PLACEMENT_3D('',#225364,#130435,#130436);
#106714=AXIS2_PLACEMENT_3D('',#225365,#130437,#130438);
#106715=AXIS2_PLACEMENT_3D('',#225366,#130439,#130440);
#106716=AXIS2_PLACEMENT_3D('',#225367,#130441,#130442);
#106717=AXIS2_PLACEMENT_3D('',#225368,#130443,#130444);
#106718=AXIS2_PLACEMENT_3D('',#225381,#130445,#130446);
#106719=AXIS2_PLACEMENT_3D('',#225382,#130447,#130448);
#106720=AXIS2_PLACEMENT_3D('',#225383,#130449,#130450);
#106721=AXIS2_PLACEMENT_3D('',#225388,#130452,#130453);
#106722=AXIS2_PLACEMENT_3D('',#225391,#130455,#130456);
#106723=AXIS2_PLACEMENT_3D('',#225392,#130457,#130458);
#106724=AXIS2_PLACEMENT_3D('',#225395,#130459,#130460);
#106725=AXIS2_PLACEMENT_3D('',#225403,#130464,#130465);
#106726=AXIS2_PLACEMENT_3D('',#225409,#130468,#130469);
#106727=AXIS2_PLACEMENT_3D('',#225413,#130471,#130472);
#106728=AXIS2_PLACEMENT_3D('',#225417,#130475,#130476);
#106729=AXIS2_PLACEMENT_3D('',#225420,#130477,#130478);
#106730=AXIS2_PLACEMENT_3D('',#225428,#130482,#130483);
#106731=AXIS2_PLACEMENT_3D('',#225434,#130486,#130487);
#106732=AXIS2_PLACEMENT_3D('',#225438,#130489,#130490);
#106733=AXIS2_PLACEMENT_3D('',#225442,#130493,#130494);
#106734=AXIS2_PLACEMENT_3D('',#225447,#130496,#130497);
#106735=AXIS2_PLACEMENT_3D('',#225450,#130499,#130500);
#106736=AXIS2_PLACEMENT_3D('',#225451,#130501,#130502);
#106737=AXIS2_PLACEMENT_3D('',#225454,#130503,#130504);
#106738=AXIS2_PLACEMENT_3D('',#225462,#130508,#130509);
#106739=AXIS2_PLACEMENT_3D('',#225468,#130512,#130513);
#106740=AXIS2_PLACEMENT_3D('',#225472,#130515,#130516);
#106741=AXIS2_PLACEMENT_3D('',#225476,#130519,#130520);
#106742=AXIS2_PLACEMENT_3D('',#225479,#130521,#130522);
#106743=AXIS2_PLACEMENT_3D('',#225487,#130526,#130527);
#106744=AXIS2_PLACEMENT_3D('',#225493,#130530,#130531);
#106745=AXIS2_PLACEMENT_3D('',#225497,#130533,#130534);
#106746=AXIS2_PLACEMENT_3D('',#225501,#130537,#130538);
#106747=AXIS2_PLACEMENT_3D('',#225506,#130540,#130541);
#106748=AXIS2_PLACEMENT_3D('',#225509,#130543,#130544);
#106749=AXIS2_PLACEMENT_3D('',#225510,#130545,#130546);
#106750=AXIS2_PLACEMENT_3D('',#225513,#130547,#130548);
#106751=AXIS2_PLACEMENT_3D('',#225521,#130552,#130553);
#106752=AXIS2_PLACEMENT_3D('',#225527,#130556,#130557);
#106753=AXIS2_PLACEMENT_3D('',#225531,#130559,#130560);
#106754=AXIS2_PLACEMENT_3D('',#225535,#130563,#130564);
#106755=AXIS2_PLACEMENT_3D('',#225538,#130565,#130566);
#106756=AXIS2_PLACEMENT_3D('',#225546,#130570,#130571);
#106757=AXIS2_PLACEMENT_3D('',#225552,#130574,#130575);
#106758=AXIS2_PLACEMENT_3D('',#225556,#130577,#130578);
#106759=AXIS2_PLACEMENT_3D('',#225560,#130581,#130582);
#106760=AXIS2_PLACEMENT_3D('',#225565,#130584,#130585);
#106761=AXIS2_PLACEMENT_3D('',#225568,#130587,#130588);
#106762=AXIS2_PLACEMENT_3D('',#225569,#130589,#130590);
#106763=AXIS2_PLACEMENT_3D('',#225572,#130591,#130592);
#106764=AXIS2_PLACEMENT_3D('',#225580,#130596,#130597);
#106765=AXIS2_PLACEMENT_3D('',#225586,#130600,#130601);
#106766=AXIS2_PLACEMENT_3D('',#225590,#130603,#130604);
#106767=AXIS2_PLACEMENT_3D('',#225594,#130607,#130608);
#106768=AXIS2_PLACEMENT_3D('',#225597,#130609,#130610);
#106769=AXIS2_PLACEMENT_3D('',#225605,#130614,#130615);
#106770=AXIS2_PLACEMENT_3D('',#225611,#130618,#130619);
#106771=AXIS2_PLACEMENT_3D('',#225615,#130621,#130622);
#106772=AXIS2_PLACEMENT_3D('',#225619,#130625,#130626);
#106773=AXIS2_PLACEMENT_3D('',#225624,#130628,#130629);
#106774=AXIS2_PLACEMENT_3D('',#225627,#130631,#130632);
#106775=AXIS2_PLACEMENT_3D('',#225628,#130633,#130634);
#106776=AXIS2_PLACEMENT_3D('',#225631,#130635,#130636);
#106777=AXIS2_PLACEMENT_3D('',#225639,#130640,#130641);
#106778=AXIS2_PLACEMENT_3D('',#225645,#130644,#130645);
#106779=AXIS2_PLACEMENT_3D('',#225649,#130647,#130648);
#106780=AXIS2_PLACEMENT_3D('',#225653,#130651,#130652);
#106781=AXIS2_PLACEMENT_3D('',#225656,#130653,#130654);
#106782=AXIS2_PLACEMENT_3D('',#225664,#130658,#130659);
#106783=AXIS2_PLACEMENT_3D('',#225670,#130662,#130663);
#106784=AXIS2_PLACEMENT_3D('',#225674,#130665,#130666);
#106785=AXIS2_PLACEMENT_3D('',#225678,#130669,#130670);
#106786=AXIS2_PLACEMENT_3D('',#225683,#130672,#130673);
#106787=AXIS2_PLACEMENT_3D('',#225686,#130675,#130676);
#106788=AXIS2_PLACEMENT_3D('',#225687,#130677,#130678);
#106789=AXIS2_PLACEMENT_3D('',#225690,#130679,#130680);
#106790=AXIS2_PLACEMENT_3D('',#225698,#130684,#130685);
#106791=AXIS2_PLACEMENT_3D('',#225704,#130688,#130689);
#106792=AXIS2_PLACEMENT_3D('',#225708,#130691,#130692);
#106793=AXIS2_PLACEMENT_3D('',#225712,#130695,#130696);
#106794=AXIS2_PLACEMENT_3D('',#225715,#130697,#130698);
#106795=AXIS2_PLACEMENT_3D('',#225723,#130702,#130703);
#106796=AXIS2_PLACEMENT_3D('',#225729,#130706,#130707);
#106797=AXIS2_PLACEMENT_3D('',#225733,#130709,#130710);
#106798=AXIS2_PLACEMENT_3D('',#225737,#130713,#130714);
#106799=AXIS2_PLACEMENT_3D('',#225742,#130716,#130717);
#106800=AXIS2_PLACEMENT_3D('',#225745,#130719,#130720);
#106801=AXIS2_PLACEMENT_3D('',#225746,#130721,#130722);
#106802=AXIS2_PLACEMENT_3D('',#225749,#130723,#130724);
#106803=AXIS2_PLACEMENT_3D('',#225757,#130728,#130729);
#106804=AXIS2_PLACEMENT_3D('',#225763,#130732,#130733);
#106805=AXIS2_PLACEMENT_3D('',#225767,#130735,#130736);
#106806=AXIS2_PLACEMENT_3D('',#225771,#130739,#130740);
#106807=AXIS2_PLACEMENT_3D('',#225774,#130741,#130742);
#106808=AXIS2_PLACEMENT_3D('',#225782,#130746,#130747);
#106809=AXIS2_PLACEMENT_3D('',#225788,#130750,#130751);
#106810=AXIS2_PLACEMENT_3D('',#225792,#130753,#130754);
#106811=AXIS2_PLACEMENT_3D('',#225796,#130757,#130758);
#106812=AXIS2_PLACEMENT_3D('',#225801,#130760,#130761);
#106813=AXIS2_PLACEMENT_3D('',#225804,#130763,#130764);
#106814=AXIS2_PLACEMENT_3D('',#225805,#130765,#130766);
#106815=AXIS2_PLACEMENT_3D('',#225808,#130767,#130768);
#106816=AXIS2_PLACEMENT_3D('',#225816,#130772,#130773);
#106817=AXIS2_PLACEMENT_3D('',#225822,#130776,#130777);
#106818=AXIS2_PLACEMENT_3D('',#225826,#130779,#130780);
#106819=AXIS2_PLACEMENT_3D('',#225830,#130783,#130784);
#106820=AXIS2_PLACEMENT_3D('',#225833,#130785,#130786);
#106821=AXIS2_PLACEMENT_3D('',#225841,#130790,#130791);
#106822=AXIS2_PLACEMENT_3D('',#225847,#130794,#130795);
#106823=AXIS2_PLACEMENT_3D('',#225851,#130797,#130798);
#106824=AXIS2_PLACEMENT_3D('',#225855,#130801,#130802);
#106825=AXIS2_PLACEMENT_3D('',#225860,#130804,#130805);
#106826=AXIS2_PLACEMENT_3D('',#225863,#130807,#130808);
#106827=AXIS2_PLACEMENT_3D('',#225864,#130809,#130810);
#106828=AXIS2_PLACEMENT_3D('',#225867,#130811,#130812);
#106829=AXIS2_PLACEMENT_3D('',#225875,#130816,#130817);
#106830=AXIS2_PLACEMENT_3D('',#225881,#130820,#130821);
#106831=AXIS2_PLACEMENT_3D('',#225885,#130823,#130824);
#106832=AXIS2_PLACEMENT_3D('',#225889,#130827,#130828);
#106833=AXIS2_PLACEMENT_3D('',#225892,#130829,#130830);
#106834=AXIS2_PLACEMENT_3D('',#225900,#130834,#130835);
#106835=AXIS2_PLACEMENT_3D('',#225906,#130838,#130839);
#106836=AXIS2_PLACEMENT_3D('',#225910,#130841,#130842);
#106837=AXIS2_PLACEMENT_3D('',#225914,#130845,#130846);
#106838=AXIS2_PLACEMENT_3D('',#225919,#130848,#130849);
#106839=AXIS2_PLACEMENT_3D('',#225922,#130851,#130852);
#106840=AXIS2_PLACEMENT_3D('',#225923,#130853,#130854);
#106841=AXIS2_PLACEMENT_3D('',#225926,#130855,#130856);
#106842=AXIS2_PLACEMENT_3D('',#225934,#130860,#130861);
#106843=AXIS2_PLACEMENT_3D('',#225940,#130864,#130865);
#106844=AXIS2_PLACEMENT_3D('',#225944,#130867,#130868);
#106845=AXIS2_PLACEMENT_3D('',#225948,#130871,#130872);
#106846=AXIS2_PLACEMENT_3D('',#225951,#130873,#130874);
#106847=AXIS2_PLACEMENT_3D('',#225959,#130878,#130879);
#106848=AXIS2_PLACEMENT_3D('',#225965,#130882,#130883);
#106849=AXIS2_PLACEMENT_3D('',#225969,#130885,#130886);
#106850=AXIS2_PLACEMENT_3D('',#225973,#130889,#130890);
#106851=AXIS2_PLACEMENT_3D('',#225978,#130892,#130893);
#106852=AXIS2_PLACEMENT_3D('',#225981,#130895,#130896);
#106853=AXIS2_PLACEMENT_3D('',#225982,#130897,#130898);
#106854=AXIS2_PLACEMENT_3D('',#225985,#130899,#130900);
#106855=AXIS2_PLACEMENT_3D('',#225993,#130904,#130905);
#106856=AXIS2_PLACEMENT_3D('',#225999,#130908,#130909);
#106857=AXIS2_PLACEMENT_3D('',#226003,#130911,#130912);
#106858=AXIS2_PLACEMENT_3D('',#226007,#130915,#130916);
#106859=AXIS2_PLACEMENT_3D('',#226010,#130917,#130918);
#106860=AXIS2_PLACEMENT_3D('',#226018,#130922,#130923);
#106861=AXIS2_PLACEMENT_3D('',#226024,#130926,#130927);
#106862=AXIS2_PLACEMENT_3D('',#226028,#130929,#130930);
#106863=AXIS2_PLACEMENT_3D('',#226032,#130933,#130934);
#106864=AXIS2_PLACEMENT_3D('',#226037,#130936,#130937);
#106865=AXIS2_PLACEMENT_3D('',#226040,#130939,#130940);
#106866=AXIS2_PLACEMENT_3D('',#226041,#130941,#130942);
#106867=AXIS2_PLACEMENT_3D('',#226044,#130943,#130944);
#106868=AXIS2_PLACEMENT_3D('',#226052,#130948,#130949);
#106869=AXIS2_PLACEMENT_3D('',#226058,#130952,#130953);
#106870=AXIS2_PLACEMENT_3D('',#226062,#130955,#130956);
#106871=AXIS2_PLACEMENT_3D('',#226066,#130959,#130960);
#106872=AXIS2_PLACEMENT_3D('',#226069,#130961,#130962);
#106873=AXIS2_PLACEMENT_3D('',#226077,#130966,#130967);
#106874=AXIS2_PLACEMENT_3D('',#226083,#130970,#130971);
#106875=AXIS2_PLACEMENT_3D('',#226087,#130973,#130974);
#106876=AXIS2_PLACEMENT_3D('',#226091,#130977,#130978);
#106877=AXIS2_PLACEMENT_3D('',#226096,#130980,#130981);
#106878=AXIS2_PLACEMENT_3D('',#226099,#130983,#130984);
#106879=AXIS2_PLACEMENT_3D('',#226100,#130985,#130986);
#106880=AXIS2_PLACEMENT_3D('',#226103,#130987,#130988);
#106881=AXIS2_PLACEMENT_3D('',#226111,#130992,#130993);
#106882=AXIS2_PLACEMENT_3D('',#226117,#130996,#130997);
#106883=AXIS2_PLACEMENT_3D('',#226121,#130999,#131000);
#106884=AXIS2_PLACEMENT_3D('',#226125,#131003,#131004);
#106885=AXIS2_PLACEMENT_3D('',#226128,#131005,#131006);
#106886=AXIS2_PLACEMENT_3D('',#226136,#131010,#131011);
#106887=AXIS2_PLACEMENT_3D('',#226142,#131014,#131015);
#106888=AXIS2_PLACEMENT_3D('',#226146,#131017,#131018);
#106889=AXIS2_PLACEMENT_3D('',#226150,#131021,#131022);
#106890=AXIS2_PLACEMENT_3D('',#226155,#131024,#131025);
#106891=AXIS2_PLACEMENT_3D('',#226158,#131027,#131028);
#106892=AXIS2_PLACEMENT_3D('',#226159,#131029,#131030);
#106893=AXIS2_PLACEMENT_3D('',#226162,#131031,#131032);
#106894=AXIS2_PLACEMENT_3D('',#226170,#131036,#131037);
#106895=AXIS2_PLACEMENT_3D('',#226176,#131040,#131041);
#106896=AXIS2_PLACEMENT_3D('',#226180,#131043,#131044);
#106897=AXIS2_PLACEMENT_3D('',#226184,#131047,#131048);
#106898=AXIS2_PLACEMENT_3D('',#226187,#131049,#131050);
#106899=AXIS2_PLACEMENT_3D('',#226195,#131054,#131055);
#106900=AXIS2_PLACEMENT_3D('',#226201,#131058,#131059);
#106901=AXIS2_PLACEMENT_3D('',#226205,#131061,#131062);
#106902=AXIS2_PLACEMENT_3D('',#226209,#131065,#131066);
#106903=AXIS2_PLACEMENT_3D('',#226214,#131068,#131069);
#106904=AXIS2_PLACEMENT_3D('',#226217,#131071,#131072);
#106905=AXIS2_PLACEMENT_3D('',#226218,#131073,#131074);
#106906=AXIS2_PLACEMENT_3D('',#226221,#131075,#131076);
#106907=AXIS2_PLACEMENT_3D('',#226229,#131080,#131081);
#106908=AXIS2_PLACEMENT_3D('',#226235,#131084,#131085);
#106909=AXIS2_PLACEMENT_3D('',#226239,#131087,#131088);
#106910=AXIS2_PLACEMENT_3D('',#226243,#131091,#131092);
#106911=AXIS2_PLACEMENT_3D('',#226246,#131093,#131094);
#106912=AXIS2_PLACEMENT_3D('',#226254,#131098,#131099);
#106913=AXIS2_PLACEMENT_3D('',#226260,#131102,#131103);
#106914=AXIS2_PLACEMENT_3D('',#226264,#131105,#131106);
#106915=AXIS2_PLACEMENT_3D('',#226268,#131109,#131110);
#106916=AXIS2_PLACEMENT_3D('',#226273,#131112,#131113);
#106917=AXIS2_PLACEMENT_3D('',#226276,#131115,#131116);
#106918=AXIS2_PLACEMENT_3D('',#226277,#131117,#131118);
#106919=AXIS2_PLACEMENT_3D('',#226280,#131119,#131120);
#106920=AXIS2_PLACEMENT_3D('',#226288,#131124,#131125);
#106921=AXIS2_PLACEMENT_3D('',#226294,#131128,#131129);
#106922=AXIS2_PLACEMENT_3D('',#226298,#131131,#131132);
#106923=AXIS2_PLACEMENT_3D('',#226302,#131135,#131136);
#106924=AXIS2_PLACEMENT_3D('',#226305,#131137,#131138);
#106925=AXIS2_PLACEMENT_3D('',#226313,#131142,#131143);
#106926=AXIS2_PLACEMENT_3D('',#226319,#131146,#131147);
#106927=AXIS2_PLACEMENT_3D('',#226323,#131149,#131150);
#106928=AXIS2_PLACEMENT_3D('',#226327,#131153,#131154);
#106929=AXIS2_PLACEMENT_3D('',#226332,#131156,#131157);
#106930=AXIS2_PLACEMENT_3D('',#226335,#131159,#131160);
#106931=AXIS2_PLACEMENT_3D('',#226336,#131161,#131162);
#106932=AXIS2_PLACEMENT_3D('',#226339,#131163,#131164);
#106933=AXIS2_PLACEMENT_3D('',#226347,#131168,#131169);
#106934=AXIS2_PLACEMENT_3D('',#226353,#131172,#131173);
#106935=AXIS2_PLACEMENT_3D('',#226357,#131175,#131176);
#106936=AXIS2_PLACEMENT_3D('',#226361,#131179,#131180);
#106937=AXIS2_PLACEMENT_3D('',#226364,#131181,#131182);
#106938=AXIS2_PLACEMENT_3D('',#226372,#131186,#131187);
#106939=AXIS2_PLACEMENT_3D('',#226378,#131190,#131191);
#106940=AXIS2_PLACEMENT_3D('',#226382,#131193,#131194);
#106941=AXIS2_PLACEMENT_3D('',#226386,#131197,#131198);
#106942=AXIS2_PLACEMENT_3D('',#226391,#131200,#131201);
#106943=AXIS2_PLACEMENT_3D('',#226394,#131203,#131204);
#106944=AXIS2_PLACEMENT_3D('',#226395,#131205,#131206);
#106945=AXIS2_PLACEMENT_3D('',#226398,#131207,#131208);
#106946=AXIS2_PLACEMENT_3D('',#226406,#131212,#131213);
#106947=AXIS2_PLACEMENT_3D('',#226412,#131216,#131217);
#106948=AXIS2_PLACEMENT_3D('',#226416,#131219,#131220);
#106949=AXIS2_PLACEMENT_3D('',#226420,#131223,#131224);
#106950=AXIS2_PLACEMENT_3D('',#226423,#131225,#131226);
#106951=AXIS2_PLACEMENT_3D('',#226431,#131230,#131231);
#106952=AXIS2_PLACEMENT_3D('',#226437,#131234,#131235);
#106953=AXIS2_PLACEMENT_3D('',#226441,#131237,#131238);
#106954=AXIS2_PLACEMENT_3D('',#226445,#131241,#131242);
#106955=AXIS2_PLACEMENT_3D('',#226450,#131244,#131245);
#106956=AXIS2_PLACEMENT_3D('',#226453,#131247,#131248);
#106957=AXIS2_PLACEMENT_3D('',#226454,#131249,#131250);
#106958=AXIS2_PLACEMENT_3D('',#226457,#131251,#131252);
#106959=AXIS2_PLACEMENT_3D('',#226465,#131256,#131257);
#106960=AXIS2_PLACEMENT_3D('',#226471,#131260,#131261);
#106961=AXIS2_PLACEMENT_3D('',#226475,#131263,#131264);
#106962=AXIS2_PLACEMENT_3D('',#226479,#131267,#131268);
#106963=AXIS2_PLACEMENT_3D('',#226482,#131269,#131270);
#106964=AXIS2_PLACEMENT_3D('',#226490,#131274,#131275);
#106965=AXIS2_PLACEMENT_3D('',#226496,#131278,#131279);
#106966=AXIS2_PLACEMENT_3D('',#226500,#131281,#131282);
#106967=AXIS2_PLACEMENT_3D('',#226504,#131285,#131286);
#106968=AXIS2_PLACEMENT_3D('',#226509,#131288,#131289);
#106969=AXIS2_PLACEMENT_3D('',#226512,#131291,#131292);
#106970=AXIS2_PLACEMENT_3D('',#226513,#131293,#131294);
#106971=AXIS2_PLACEMENT_3D('',#226516,#131295,#131296);
#106972=AXIS2_PLACEMENT_3D('',#226524,#131300,#131301);
#106973=AXIS2_PLACEMENT_3D('',#226530,#131304,#131305);
#106974=AXIS2_PLACEMENT_3D('',#226534,#131307,#131308);
#106975=AXIS2_PLACEMENT_3D('',#226538,#131311,#131312);
#106976=AXIS2_PLACEMENT_3D('',#226541,#131313,#131314);
#106977=AXIS2_PLACEMENT_3D('',#226549,#131318,#131319);
#106978=AXIS2_PLACEMENT_3D('',#226555,#131322,#131323);
#106979=AXIS2_PLACEMENT_3D('',#226559,#131325,#131326);
#106980=AXIS2_PLACEMENT_3D('',#226563,#131329,#131330);
#106981=AXIS2_PLACEMENT_3D('',#226568,#131332,#131333);
#106982=AXIS2_PLACEMENT_3D('',#226571,#131335,#131336);
#106983=AXIS2_PLACEMENT_3D('',#226572,#131337,#131338);
#106984=AXIS2_PLACEMENT_3D('',#226575,#131339,#131340);
#106985=AXIS2_PLACEMENT_3D('',#226583,#131344,#131345);
#106986=AXIS2_PLACEMENT_3D('',#226589,#131348,#131349);
#106987=AXIS2_PLACEMENT_3D('',#226593,#131351,#131352);
#106988=AXIS2_PLACEMENT_3D('',#226597,#131355,#131356);
#106989=AXIS2_PLACEMENT_3D('',#226600,#131357,#131358);
#106990=AXIS2_PLACEMENT_3D('',#226608,#131362,#131363);
#106991=AXIS2_PLACEMENT_3D('',#226614,#131366,#131367);
#106992=AXIS2_PLACEMENT_3D('',#226618,#131369,#131370);
#106993=AXIS2_PLACEMENT_3D('',#226622,#131373,#131374);
#106994=AXIS2_PLACEMENT_3D('',#226627,#131376,#131377);
#106995=AXIS2_PLACEMENT_3D('',#226630,#131379,#131380);
#106996=AXIS2_PLACEMENT_3D('',#226631,#131381,#131382);
#106997=AXIS2_PLACEMENT_3D('',#226634,#131383,#131384);
#106998=AXIS2_PLACEMENT_3D('',#226642,#131388,#131389);
#106999=AXIS2_PLACEMENT_3D('',#226648,#131392,#131393);
#107000=AXIS2_PLACEMENT_3D('',#226652,#131395,#131396);
#107001=AXIS2_PLACEMENT_3D('',#226656,#131399,#131400);
#107002=AXIS2_PLACEMENT_3D('',#226659,#131401,#131402);
#107003=AXIS2_PLACEMENT_3D('',#226667,#131406,#131407);
#107004=AXIS2_PLACEMENT_3D('',#226673,#131410,#131411);
#107005=AXIS2_PLACEMENT_3D('',#226677,#131413,#131414);
#107006=AXIS2_PLACEMENT_3D('',#226681,#131417,#131418);
#107007=AXIS2_PLACEMENT_3D('',#226686,#131420,#131421);
#107008=AXIS2_PLACEMENT_3D('',#226689,#131423,#131424);
#107009=AXIS2_PLACEMENT_3D('',#226690,#131425,#131426);
#107010=AXIS2_PLACEMENT_3D('',#226693,#131427,#131428);
#107011=AXIS2_PLACEMENT_3D('',#226701,#131432,#131433);
#107012=AXIS2_PLACEMENT_3D('',#226707,#131436,#131437);
#107013=AXIS2_PLACEMENT_3D('',#226711,#131439,#131440);
#107014=AXIS2_PLACEMENT_3D('',#226715,#131443,#131444);
#107015=AXIS2_PLACEMENT_3D('',#226718,#131445,#131446);
#107016=AXIS2_PLACEMENT_3D('',#226726,#131450,#131451);
#107017=AXIS2_PLACEMENT_3D('',#226732,#131454,#131455);
#107018=AXIS2_PLACEMENT_3D('',#226736,#131457,#131458);
#107019=AXIS2_PLACEMENT_3D('',#226740,#131461,#131462);
#107020=AXIS2_PLACEMENT_3D('',#226745,#131464,#131465);
#107021=AXIS2_PLACEMENT_3D('',#226748,#131467,#131468);
#107022=AXIS2_PLACEMENT_3D('',#226749,#131469,#131470);
#107023=AXIS2_PLACEMENT_3D('',#226752,#131471,#131472);
#107024=AXIS2_PLACEMENT_3D('',#226760,#131476,#131477);
#107025=AXIS2_PLACEMENT_3D('',#226766,#131480,#131481);
#107026=AXIS2_PLACEMENT_3D('',#226770,#131483,#131484);
#107027=AXIS2_PLACEMENT_3D('',#226774,#131487,#131488);
#107028=AXIS2_PLACEMENT_3D('',#226777,#131489,#131490);
#107029=AXIS2_PLACEMENT_3D('',#226785,#131494,#131495);
#107030=AXIS2_PLACEMENT_3D('',#226791,#131498,#131499);
#107031=AXIS2_PLACEMENT_3D('',#226795,#131501,#131502);
#107032=AXIS2_PLACEMENT_3D('',#226799,#131505,#131506);
#107033=AXIS2_PLACEMENT_3D('',#226804,#131508,#131509);
#107034=AXIS2_PLACEMENT_3D('',#226807,#131511,#131512);
#107035=AXIS2_PLACEMENT_3D('',#226808,#131513,#131514);
#107036=AXIS2_PLACEMENT_3D('',#226811,#131515,#131516);
#107037=AXIS2_PLACEMENT_3D('',#226819,#131520,#131521);
#107038=AXIS2_PLACEMENT_3D('',#226825,#131524,#131525);
#107039=AXIS2_PLACEMENT_3D('',#226829,#131527,#131528);
#107040=AXIS2_PLACEMENT_3D('',#226833,#131531,#131532);
#107041=AXIS2_PLACEMENT_3D('',#226836,#131533,#131534);
#107042=AXIS2_PLACEMENT_3D('',#226844,#131538,#131539);
#107043=AXIS2_PLACEMENT_3D('',#226850,#131542,#131543);
#107044=AXIS2_PLACEMENT_3D('',#226854,#131545,#131546);
#107045=AXIS2_PLACEMENT_3D('',#226858,#131549,#131550);
#107046=AXIS2_PLACEMENT_3D('',#226863,#131552,#131553);
#107047=AXIS2_PLACEMENT_3D('',#226866,#131555,#131556);
#107048=AXIS2_PLACEMENT_3D('',#226867,#131557,#131558);
#107049=AXIS2_PLACEMENT_3D('',#226870,#131559,#131560);
#107050=AXIS2_PLACEMENT_3D('',#226878,#131564,#131565);
#107051=AXIS2_PLACEMENT_3D('',#226884,#131568,#131569);
#107052=AXIS2_PLACEMENT_3D('',#226888,#131571,#131572);
#107053=AXIS2_PLACEMENT_3D('',#226892,#131575,#131576);
#107054=AXIS2_PLACEMENT_3D('',#226895,#131577,#131578);
#107055=AXIS2_PLACEMENT_3D('',#226903,#131582,#131583);
#107056=AXIS2_PLACEMENT_3D('',#226909,#131586,#131587);
#107057=AXIS2_PLACEMENT_3D('',#226913,#131589,#131590);
#107058=AXIS2_PLACEMENT_3D('',#226917,#131593,#131594);
#107059=AXIS2_PLACEMENT_3D('',#226922,#131596,#131597);
#107060=AXIS2_PLACEMENT_3D('',#226925,#131599,#131600);
#107061=AXIS2_PLACEMENT_3D('',#226926,#131601,#131602);
#107062=AXIS2_PLACEMENT_3D('',#226929,#131603,#131604);
#107063=AXIS2_PLACEMENT_3D('',#226937,#131608,#131609);
#107064=AXIS2_PLACEMENT_3D('',#226943,#131612,#131613);
#107065=AXIS2_PLACEMENT_3D('',#226947,#131615,#131616);
#107066=AXIS2_PLACEMENT_3D('',#226951,#131619,#131620);
#107067=AXIS2_PLACEMENT_3D('',#226954,#131621,#131622);
#107068=AXIS2_PLACEMENT_3D('',#226962,#131626,#131627);
#107069=AXIS2_PLACEMENT_3D('',#226968,#131630,#131631);
#107070=AXIS2_PLACEMENT_3D('',#226972,#131633,#131634);
#107071=AXIS2_PLACEMENT_3D('',#226976,#131637,#131638);
#107072=AXIS2_PLACEMENT_3D('',#226981,#131640,#131641);
#107073=AXIS2_PLACEMENT_3D('',#226984,#131643,#131644);
#107074=AXIS2_PLACEMENT_3D('',#226985,#131645,#131646);
#107075=AXIS2_PLACEMENT_3D('',#226988,#131647,#131648);
#107076=AXIS2_PLACEMENT_3D('',#226996,#131652,#131653);
#107077=AXIS2_PLACEMENT_3D('',#227002,#131656,#131657);
#107078=AXIS2_PLACEMENT_3D('',#227006,#131659,#131660);
#107079=AXIS2_PLACEMENT_3D('',#227010,#131663,#131664);
#107080=AXIS2_PLACEMENT_3D('',#227013,#131665,#131666);
#107081=AXIS2_PLACEMENT_3D('',#227021,#131670,#131671);
#107082=AXIS2_PLACEMENT_3D('',#227027,#131674,#131675);
#107083=AXIS2_PLACEMENT_3D('',#227031,#131677,#131678);
#107084=AXIS2_PLACEMENT_3D('',#227035,#131681,#131682);
#107085=AXIS2_PLACEMENT_3D('',#227040,#131684,#131685);
#107086=AXIS2_PLACEMENT_3D('',#227043,#131687,#131688);
#107087=AXIS2_PLACEMENT_3D('',#227044,#131689,#131690);
#107088=AXIS2_PLACEMENT_3D('',#227047,#131691,#131692);
#107089=AXIS2_PLACEMENT_3D('',#227055,#131696,#131697);
#107090=AXIS2_PLACEMENT_3D('',#227061,#131700,#131701);
#107091=AXIS2_PLACEMENT_3D('',#227065,#131703,#131704);
#107092=AXIS2_PLACEMENT_3D('',#227069,#131707,#131708);
#107093=AXIS2_PLACEMENT_3D('',#227072,#131709,#131710);
#107094=AXIS2_PLACEMENT_3D('',#227080,#131714,#131715);
#107095=AXIS2_PLACEMENT_3D('',#227086,#131718,#131719);
#107096=AXIS2_PLACEMENT_3D('',#227090,#131721,#131722);
#107097=AXIS2_PLACEMENT_3D('',#227094,#131725,#131726);
#107098=AXIS2_PLACEMENT_3D('',#227097,#131729,#131730);
#107099=AXIS2_PLACEMENT_3D('',#227100,#131731,#131732);
#107100=AXIS2_PLACEMENT_3D('',#227108,#131736,#131737);
#107101=AXIS2_PLACEMENT_3D('',#227114,#131740,#131741);
#107102=AXIS2_PLACEMENT_3D('',#227118,#131743,#131744);
#107103=AXIS2_PLACEMENT_3D('',#227122,#131747,#131748);
#107104=AXIS2_PLACEMENT_3D('',#227125,#131749,#131750);
#107105=AXIS2_PLACEMENT_3D('',#227133,#131754,#131755);
#107106=AXIS2_PLACEMENT_3D('',#227139,#131758,#131759);
#107107=AXIS2_PLACEMENT_3D('',#227143,#131761,#131762);
#107108=AXIS2_PLACEMENT_3D('',#227147,#131765,#131766);
#107109=AXIS2_PLACEMENT_3D('',#227152,#131768,#131769);
#107110=AXIS2_PLACEMENT_3D('',#227155,#131771,#131772);
#107111=AXIS2_PLACEMENT_3D('',#227156,#131773,#131774);
#107112=AXIS2_PLACEMENT_3D('',#227159,#131775,#131776);
#107113=AXIS2_PLACEMENT_3D('',#227167,#131780,#131781);
#107114=AXIS2_PLACEMENT_3D('',#227173,#131784,#131785);
#107115=AXIS2_PLACEMENT_3D('',#227177,#131787,#131788);
#107116=AXIS2_PLACEMENT_3D('',#227181,#131791,#131792);
#107117=AXIS2_PLACEMENT_3D('',#227184,#131793,#131794);
#107118=AXIS2_PLACEMENT_3D('',#227192,#131798,#131799);
#107119=AXIS2_PLACEMENT_3D('',#227198,#131802,#131803);
#107120=AXIS2_PLACEMENT_3D('',#227202,#131805,#131806);
#107121=AXIS2_PLACEMENT_3D('',#227206,#131809,#131810);
#107122=AXIS2_PLACEMENT_3D('',#227211,#131812,#131813);
#107123=AXIS2_PLACEMENT_3D('',#227214,#131815,#131816);
#107124=AXIS2_PLACEMENT_3D('',#227215,#131817,#131818);
#107125=AXIS2_PLACEMENT_3D('',#227218,#131819,#131820);
#107126=AXIS2_PLACEMENT_3D('',#227226,#131824,#131825);
#107127=AXIS2_PLACEMENT_3D('',#227232,#131828,#131829);
#107128=AXIS2_PLACEMENT_3D('',#227236,#131831,#131832);
#107129=AXIS2_PLACEMENT_3D('',#227240,#131835,#131836);
#107130=AXIS2_PLACEMENT_3D('',#227243,#131837,#131838);
#107131=AXIS2_PLACEMENT_3D('',#227251,#131842,#131843);
#107132=AXIS2_PLACEMENT_3D('',#227257,#131846,#131847);
#107133=AXIS2_PLACEMENT_3D('',#227261,#131849,#131850);
#107134=AXIS2_PLACEMENT_3D('',#227265,#131853,#131854);
#107135=AXIS2_PLACEMENT_3D('',#227270,#131856,#131857);
#107136=AXIS2_PLACEMENT_3D('',#227273,#131859,#131860);
#107137=AXIS2_PLACEMENT_3D('',#227274,#131861,#131862);
#107138=AXIS2_PLACEMENT_3D('',#227277,#131863,#131864);
#107139=AXIS2_PLACEMENT_3D('',#227285,#131868,#131869);
#107140=AXIS2_PLACEMENT_3D('',#227291,#131872,#131873);
#107141=AXIS2_PLACEMENT_3D('',#227295,#131875,#131876);
#107142=AXIS2_PLACEMENT_3D('',#227299,#131879,#131880);
#107143=AXIS2_PLACEMENT_3D('',#227302,#131881,#131882);
#107144=AXIS2_PLACEMENT_3D('',#227310,#131886,#131887);
#107145=AXIS2_PLACEMENT_3D('',#227316,#131890,#131891);
#107146=AXIS2_PLACEMENT_3D('',#227320,#131893,#131894);
#107147=AXIS2_PLACEMENT_3D('',#227324,#131897,#131898);
#107148=AXIS2_PLACEMENT_3D('',#227329,#131900,#131901);
#107149=AXIS2_PLACEMENT_3D('',#227332,#131903,#131904);
#107150=AXIS2_PLACEMENT_3D('',#227333,#131905,#131906);
#107151=AXIS2_PLACEMENT_3D('',#227336,#131907,#131908);
#107152=AXIS2_PLACEMENT_3D('',#227344,#131912,#131913);
#107153=AXIS2_PLACEMENT_3D('',#227350,#131916,#131917);
#107154=AXIS2_PLACEMENT_3D('',#227354,#131919,#131920);
#107155=AXIS2_PLACEMENT_3D('',#227358,#131923,#131924);
#107156=AXIS2_PLACEMENT_3D('',#227361,#131925,#131926);
#107157=AXIS2_PLACEMENT_3D('',#227369,#131930,#131931);
#107158=AXIS2_PLACEMENT_3D('',#227375,#131934,#131935);
#107159=AXIS2_PLACEMENT_3D('',#227379,#131937,#131938);
#107160=AXIS2_PLACEMENT_3D('',#227383,#131941,#131942);
#107161=AXIS2_PLACEMENT_3D('',#227388,#131944,#131945);
#107162=AXIS2_PLACEMENT_3D('',#227391,#131947,#131948);
#107163=AXIS2_PLACEMENT_3D('',#227392,#131949,#131950);
#107164=AXIS2_PLACEMENT_3D('',#227395,#131951,#131952);
#107165=AXIS2_PLACEMENT_3D('',#227403,#131956,#131957);
#107166=AXIS2_PLACEMENT_3D('',#227409,#131960,#131961);
#107167=AXIS2_PLACEMENT_3D('',#227413,#131963,#131964);
#107168=AXIS2_PLACEMENT_3D('',#227417,#131967,#131968);
#107169=AXIS2_PLACEMENT_3D('',#227420,#131969,#131970);
#107170=AXIS2_PLACEMENT_3D('',#227428,#131974,#131975);
#107171=AXIS2_PLACEMENT_3D('',#227434,#131978,#131979);
#107172=AXIS2_PLACEMENT_3D('',#227438,#131981,#131982);
#107173=AXIS2_PLACEMENT_3D('',#227442,#131985,#131986);
#107174=AXIS2_PLACEMENT_3D('',#227447,#131988,#131989);
#107175=AXIS2_PLACEMENT_3D('',#227450,#131991,#131992);
#107176=AXIS2_PLACEMENT_3D('',#227451,#131993,#131994);
#107177=AXIS2_PLACEMENT_3D('',#227454,#131995,#131996);
#107178=AXIS2_PLACEMENT_3D('',#227462,#132000,#132001);
#107179=AXIS2_PLACEMENT_3D('',#227468,#132004,#132005);
#107180=AXIS2_PLACEMENT_3D('',#227472,#132007,#132008);
#107181=AXIS2_PLACEMENT_3D('',#227476,#132011,#132012);
#107182=AXIS2_PLACEMENT_3D('',#227479,#132013,#132014);
#107183=AXIS2_PLACEMENT_3D('',#227487,#132018,#132019);
#107184=AXIS2_PLACEMENT_3D('',#227493,#132022,#132023);
#107185=AXIS2_PLACEMENT_3D('',#227497,#132025,#132026);
#107186=AXIS2_PLACEMENT_3D('',#227501,#132029,#132030);
#107187=AXIS2_PLACEMENT_3D('',#227506,#132032,#132033);
#107188=AXIS2_PLACEMENT_3D('',#227509,#132035,#132036);
#107189=AXIS2_PLACEMENT_3D('',#227510,#132037,#132038);
#107190=AXIS2_PLACEMENT_3D('',#227513,#132039,#132040);
#107191=AXIS2_PLACEMENT_3D('',#227521,#132044,#132045);
#107192=AXIS2_PLACEMENT_3D('',#227527,#132048,#132049);
#107193=AXIS2_PLACEMENT_3D('',#227531,#132051,#132052);
#107194=AXIS2_PLACEMENT_3D('',#227535,#132055,#132056);
#107195=AXIS2_PLACEMENT_3D('',#227538,#132057,#132058);
#107196=AXIS2_PLACEMENT_3D('',#227546,#132062,#132063);
#107197=AXIS2_PLACEMENT_3D('',#227552,#132066,#132067);
#107198=AXIS2_PLACEMENT_3D('',#227556,#132069,#132070);
#107199=AXIS2_PLACEMENT_3D('',#227560,#132073,#132074);
#107200=AXIS2_PLACEMENT_3D('',#227565,#132076,#132077);
#107201=AXIS2_PLACEMENT_3D('',#227568,#132079,#132080);
#107202=AXIS2_PLACEMENT_3D('',#227569,#132081,#132082);
#107203=AXIS2_PLACEMENT_3D('',#227572,#132083,#132084);
#107204=AXIS2_PLACEMENT_3D('',#227580,#132088,#132089);
#107205=AXIS2_PLACEMENT_3D('',#227586,#132092,#132093);
#107206=AXIS2_PLACEMENT_3D('',#227590,#132095,#132096);
#107207=AXIS2_PLACEMENT_3D('',#227594,#132099,#132100);
#107208=AXIS2_PLACEMENT_3D('',#227597,#132101,#132102);
#107209=AXIS2_PLACEMENT_3D('',#227605,#132106,#132107);
#107210=AXIS2_PLACEMENT_3D('',#227611,#132110,#132111);
#107211=AXIS2_PLACEMENT_3D('',#227615,#132113,#132114);
#107212=AXIS2_PLACEMENT_3D('',#227619,#132117,#132118);
#107213=AXIS2_PLACEMENT_3D('',#227624,#132120,#132121);
#107214=AXIS2_PLACEMENT_3D('',#227627,#132123,#132124);
#107215=AXIS2_PLACEMENT_3D('',#227628,#132125,#132126);
#107216=AXIS2_PLACEMENT_3D('',#227631,#132127,#132128);
#107217=AXIS2_PLACEMENT_3D('',#227639,#132132,#132133);
#107218=AXIS2_PLACEMENT_3D('',#227645,#132136,#132137);
#107219=AXIS2_PLACEMENT_3D('',#227649,#132139,#132140);
#107220=AXIS2_PLACEMENT_3D('',#227653,#132143,#132144);
#107221=AXIS2_PLACEMENT_3D('',#227656,#132145,#132146);
#107222=AXIS2_PLACEMENT_3D('',#227664,#132150,#132151);
#107223=AXIS2_PLACEMENT_3D('',#227670,#132154,#132155);
#107224=AXIS2_PLACEMENT_3D('',#227674,#132157,#132158);
#107225=AXIS2_PLACEMENT_3D('',#227678,#132161,#132162);
#107226=AXIS2_PLACEMENT_3D('',#227683,#132164,#132165);
#107227=AXIS2_PLACEMENT_3D('',#227686,#132167,#132168);
#107228=AXIS2_PLACEMENT_3D('',#227687,#132169,#132170);
#107229=AXIS2_PLACEMENT_3D('',#227690,#132171,#132172);
#107230=AXIS2_PLACEMENT_3D('',#227698,#132176,#132177);
#107231=AXIS2_PLACEMENT_3D('',#227704,#132180,#132181);
#107232=AXIS2_PLACEMENT_3D('',#227708,#132183,#132184);
#107233=AXIS2_PLACEMENT_3D('',#227712,#132187,#132188);
#107234=AXIS2_PLACEMENT_3D('',#227715,#132189,#132190);
#107235=AXIS2_PLACEMENT_3D('',#227723,#132194,#132195);
#107236=AXIS2_PLACEMENT_3D('',#227729,#132198,#132199);
#107237=AXIS2_PLACEMENT_3D('',#227733,#132201,#132202);
#107238=AXIS2_PLACEMENT_3D('',#227737,#132205,#132206);
#107239=AXIS2_PLACEMENT_3D('',#227742,#132208,#132209);
#107240=AXIS2_PLACEMENT_3D('',#227745,#132211,#132212);
#107241=AXIS2_PLACEMENT_3D('',#227746,#132213,#132214);
#107242=AXIS2_PLACEMENT_3D('',#227749,#132215,#132216);
#107243=AXIS2_PLACEMENT_3D('',#227757,#132220,#132221);
#107244=AXIS2_PLACEMENT_3D('',#227763,#132224,#132225);
#107245=AXIS2_PLACEMENT_3D('',#227767,#132227,#132228);
#107246=AXIS2_PLACEMENT_3D('',#227771,#132231,#132232);
#107247=AXIS2_PLACEMENT_3D('',#227774,#132233,#132234);
#107248=AXIS2_PLACEMENT_3D('',#227782,#132238,#132239);
#107249=AXIS2_PLACEMENT_3D('',#227788,#132242,#132243);
#107250=AXIS2_PLACEMENT_3D('',#227792,#132245,#132246);
#107251=AXIS2_PLACEMENT_3D('',#227796,#132249,#132250);
#107252=AXIS2_PLACEMENT_3D('',#227801,#132252,#132253);
#107253=AXIS2_PLACEMENT_3D('',#227804,#132255,#132256);
#107254=AXIS2_PLACEMENT_3D('',#227805,#132257,#132258);
#107255=AXIS2_PLACEMENT_3D('',#227808,#132259,#132260);
#107256=AXIS2_PLACEMENT_3D('',#227816,#132264,#132265);
#107257=AXIS2_PLACEMENT_3D('',#227822,#132268,#132269);
#107258=AXIS2_PLACEMENT_3D('',#227826,#132271,#132272);
#107259=AXIS2_PLACEMENT_3D('',#227830,#132275,#132276);
#107260=AXIS2_PLACEMENT_3D('',#227833,#132277,#132278);
#107261=AXIS2_PLACEMENT_3D('',#227841,#132282,#132283);
#107262=AXIS2_PLACEMENT_3D('',#227847,#132286,#132287);
#107263=AXIS2_PLACEMENT_3D('',#227851,#132289,#132290);
#107264=AXIS2_PLACEMENT_3D('',#227855,#132293,#132294);
#107265=AXIS2_PLACEMENT_3D('',#227860,#132296,#132297);
#107266=AXIS2_PLACEMENT_3D('',#227863,#132299,#132300);
#107267=AXIS2_PLACEMENT_3D('',#227864,#132301,#132302);
#107268=AXIS2_PLACEMENT_3D('',#227867,#132303,#132304);
#107269=AXIS2_PLACEMENT_3D('',#227875,#132308,#132309);
#107270=AXIS2_PLACEMENT_3D('',#227881,#132312,#132313);
#107271=AXIS2_PLACEMENT_3D('',#227885,#132315,#132316);
#107272=AXIS2_PLACEMENT_3D('',#227889,#132319,#132320);
#107273=AXIS2_PLACEMENT_3D('',#227892,#132321,#132322);
#107274=AXIS2_PLACEMENT_3D('',#227900,#132326,#132327);
#107275=AXIS2_PLACEMENT_3D('',#227906,#132330,#132331);
#107276=AXIS2_PLACEMENT_3D('',#227910,#132333,#132334);
#107277=AXIS2_PLACEMENT_3D('',#227914,#132337,#132338);
#107278=AXIS2_PLACEMENT_3D('',#227919,#132340,#132341);
#107279=AXIS2_PLACEMENT_3D('',#227922,#132343,#132344);
#107280=AXIS2_PLACEMENT_3D('',#227923,#132345,#132346);
#107281=AXIS2_PLACEMENT_3D('',#227926,#132347,#132348);
#107282=AXIS2_PLACEMENT_3D('',#227934,#132352,#132353);
#107283=AXIS2_PLACEMENT_3D('',#227940,#132356,#132357);
#107284=AXIS2_PLACEMENT_3D('',#227944,#132359,#132360);
#107285=AXIS2_PLACEMENT_3D('',#227948,#132363,#132364);
#107286=AXIS2_PLACEMENT_3D('',#227951,#132365,#132366);
#107287=AXIS2_PLACEMENT_3D('',#227959,#132370,#132371);
#107288=AXIS2_PLACEMENT_3D('',#227965,#132374,#132375);
#107289=AXIS2_PLACEMENT_3D('',#227969,#132377,#132378);
#107290=AXIS2_PLACEMENT_3D('',#227973,#132381,#132382);
#107291=AXIS2_PLACEMENT_3D('',#227976,#132385,#132386);
#107292=AXIS2_PLACEMENT_3D('',#227979,#132387,#132388);
#107293=AXIS2_PLACEMENT_3D('',#227987,#132392,#132393);
#107294=AXIS2_PLACEMENT_3D('',#227993,#132396,#132397);
#107295=AXIS2_PLACEMENT_3D('',#227997,#132399,#132400);
#107296=AXIS2_PLACEMENT_3D('',#228001,#132403,#132404);
#107297=AXIS2_PLACEMENT_3D('',#228004,#132405,#132406);
#107298=AXIS2_PLACEMENT_3D('',#228012,#132410,#132411);
#107299=AXIS2_PLACEMENT_3D('',#228018,#132414,#132415);
#107300=AXIS2_PLACEMENT_3D('',#228022,#132417,#132418);
#107301=AXIS2_PLACEMENT_3D('',#228026,#132421,#132422);
#107302=AXIS2_PLACEMENT_3D('',#228031,#132424,#132425);
#107303=AXIS2_PLACEMENT_3D('',#228034,#132427,#132428);
#107304=AXIS2_PLACEMENT_3D('',#228035,#132429,#132430);
#107305=AXIS2_PLACEMENT_3D('',#228038,#132431,#132432);
#107306=AXIS2_PLACEMENT_3D('',#228046,#132436,#132437);
#107307=AXIS2_PLACEMENT_3D('',#228052,#132440,#132441);
#107308=AXIS2_PLACEMENT_3D('',#228056,#132443,#132444);
#107309=AXIS2_PLACEMENT_3D('',#228060,#132447,#132448);
#107310=AXIS2_PLACEMENT_3D('',#228063,#132449,#132450);
#107311=AXIS2_PLACEMENT_3D('',#228071,#132454,#132455);
#107312=AXIS2_PLACEMENT_3D('',#228077,#132458,#132459);
#107313=AXIS2_PLACEMENT_3D('',#228081,#132461,#132462);
#107314=AXIS2_PLACEMENT_3D('',#228085,#132465,#132466);
#107315=AXIS2_PLACEMENT_3D('',#228090,#132468,#132469);
#107316=AXIS2_PLACEMENT_3D('',#228093,#132471,#132472);
#107317=AXIS2_PLACEMENT_3D('',#228094,#132473,#132474);
#107318=AXIS2_PLACEMENT_3D('',#228097,#132475,#132476);
#107319=AXIS2_PLACEMENT_3D('',#228105,#132480,#132481);
#107320=AXIS2_PLACEMENT_3D('',#228111,#132484,#132485);
#107321=AXIS2_PLACEMENT_3D('',#228115,#132487,#132488);
#107322=AXIS2_PLACEMENT_3D('',#228119,#132491,#132492);
#107323=AXIS2_PLACEMENT_3D('',#228122,#132493,#132494);
#107324=AXIS2_PLACEMENT_3D('',#228130,#132498,#132499);
#107325=AXIS2_PLACEMENT_3D('',#228136,#132502,#132503);
#107326=AXIS2_PLACEMENT_3D('',#228140,#132505,#132506);
#107327=AXIS2_PLACEMENT_3D('',#228144,#132509,#132510);
#107328=AXIS2_PLACEMENT_3D('',#228149,#132512,#132513);
#107329=AXIS2_PLACEMENT_3D('',#228152,#132515,#132516);
#107330=AXIS2_PLACEMENT_3D('',#228153,#132517,#132518);
#107331=AXIS2_PLACEMENT_3D('',#228156,#132519,#132520);
#107332=AXIS2_PLACEMENT_3D('',#228164,#132524,#132525);
#107333=AXIS2_PLACEMENT_3D('',#228170,#132528,#132529);
#107334=AXIS2_PLACEMENT_3D('',#228174,#132531,#132532);
#107335=AXIS2_PLACEMENT_3D('',#228178,#132535,#132536);
#107336=AXIS2_PLACEMENT_3D('',#228181,#132537,#132538);
#107337=AXIS2_PLACEMENT_3D('',#228189,#132542,#132543);
#107338=AXIS2_PLACEMENT_3D('',#228195,#132546,#132547);
#107339=AXIS2_PLACEMENT_3D('',#228199,#132549,#132550);
#107340=AXIS2_PLACEMENT_3D('',#228203,#132553,#132554);
#107341=AXIS2_PLACEMENT_3D('',#228208,#132556,#132557);
#107342=AXIS2_PLACEMENT_3D('',#228211,#132559,#132560);
#107343=AXIS2_PLACEMENT_3D('',#228212,#132561,#132562);
#107344=AXIS2_PLACEMENT_3D('',#228215,#132563,#132564);
#107345=AXIS2_PLACEMENT_3D('',#228223,#132568,#132569);
#107346=AXIS2_PLACEMENT_3D('',#228229,#132572,#132573);
#107347=AXIS2_PLACEMENT_3D('',#228233,#132575,#132576);
#107348=AXIS2_PLACEMENT_3D('',#228237,#132579,#132580);
#107349=AXIS2_PLACEMENT_3D('',#228240,#132581,#132582);
#107350=AXIS2_PLACEMENT_3D('',#228248,#132586,#132587);
#107351=AXIS2_PLACEMENT_3D('',#228254,#132590,#132591);
#107352=AXIS2_PLACEMENT_3D('',#228258,#132593,#132594);
#107353=AXIS2_PLACEMENT_3D('',#228262,#132597,#132598);
#107354=AXIS2_PLACEMENT_3D('',#228267,#132600,#132601);
#107355=AXIS2_PLACEMENT_3D('',#228270,#132603,#132604);
#107356=AXIS2_PLACEMENT_3D('',#228271,#132605,#132606);
#107357=AXIS2_PLACEMENT_3D('',#228274,#132607,#132608);
#107358=AXIS2_PLACEMENT_3D('',#228282,#132612,#132613);
#107359=AXIS2_PLACEMENT_3D('',#228288,#132616,#132617);
#107360=AXIS2_PLACEMENT_3D('',#228292,#132619,#132620);
#107361=AXIS2_PLACEMENT_3D('',#228296,#132623,#132624);
#107362=AXIS2_PLACEMENT_3D('',#228299,#132625,#132626);
#107363=AXIS2_PLACEMENT_3D('',#228307,#132630,#132631);
#107364=AXIS2_PLACEMENT_3D('',#228313,#132634,#132635);
#107365=AXIS2_PLACEMENT_3D('',#228317,#132637,#132638);
#107366=AXIS2_PLACEMENT_3D('',#228321,#132641,#132642);
#107367=AXIS2_PLACEMENT_3D('',#228326,#132644,#132645);
#107368=AXIS2_PLACEMENT_3D('',#228329,#132647,#132648);
#107369=AXIS2_PLACEMENT_3D('',#228330,#132649,#132650);
#107370=AXIS2_PLACEMENT_3D('',#228333,#132651,#132652);
#107371=AXIS2_PLACEMENT_3D('',#228341,#132656,#132657);
#107372=AXIS2_PLACEMENT_3D('',#228347,#132660,#132661);
#107373=AXIS2_PLACEMENT_3D('',#228351,#132663,#132664);
#107374=AXIS2_PLACEMENT_3D('',#228355,#132667,#132668);
#107375=AXIS2_PLACEMENT_3D('',#228358,#132669,#132670);
#107376=AXIS2_PLACEMENT_3D('',#228366,#132674,#132675);
#107377=AXIS2_PLACEMENT_3D('',#228372,#132678,#132679);
#107378=AXIS2_PLACEMENT_3D('',#228376,#132681,#132682);
#107379=AXIS2_PLACEMENT_3D('',#228380,#132685,#132686);
#107380=AXIS2_PLACEMENT_3D('',#228385,#132688,#132689);
#107381=AXIS2_PLACEMENT_3D('',#228388,#132691,#132692);
#107382=AXIS2_PLACEMENT_3D('',#228389,#132693,#132694);
#107383=AXIS2_PLACEMENT_3D('',#228392,#132695,#132696);
#107384=AXIS2_PLACEMENT_3D('',#228400,#132700,#132701);
#107385=AXIS2_PLACEMENT_3D('',#228406,#132704,#132705);
#107386=AXIS2_PLACEMENT_3D('',#228410,#132707,#132708);
#107387=AXIS2_PLACEMENT_3D('',#228414,#132711,#132712);
#107388=AXIS2_PLACEMENT_3D('',#228417,#132713,#132714);
#107389=AXIS2_PLACEMENT_3D('',#228425,#132718,#132719);
#107390=AXIS2_PLACEMENT_3D('',#228431,#132722,#132723);
#107391=AXIS2_PLACEMENT_3D('',#228435,#132725,#132726);
#107392=AXIS2_PLACEMENT_3D('',#228439,#132729,#132730);
#107393=AXIS2_PLACEMENT_3D('',#228444,#132732,#132733);
#107394=AXIS2_PLACEMENT_3D('',#228447,#132735,#132736);
#107395=AXIS2_PLACEMENT_3D('',#228448,#132737,#132738);
#107396=AXIS2_PLACEMENT_3D('',#228451,#132739,#132740);
#107397=AXIS2_PLACEMENT_3D('',#228459,#132744,#132745);
#107398=AXIS2_PLACEMENT_3D('',#228465,#132748,#132749);
#107399=AXIS2_PLACEMENT_3D('',#228469,#132751,#132752);
#107400=AXIS2_PLACEMENT_3D('',#228473,#132755,#132756);
#107401=AXIS2_PLACEMENT_3D('',#228476,#132757,#132758);
#107402=AXIS2_PLACEMENT_3D('',#228484,#132762,#132763);
#107403=AXIS2_PLACEMENT_3D('',#228490,#132766,#132767);
#107404=AXIS2_PLACEMENT_3D('',#228494,#132769,#132770);
#107405=AXIS2_PLACEMENT_3D('',#228498,#132773,#132774);
#107406=AXIS2_PLACEMENT_3D('',#228503,#132776,#132777);
#107407=AXIS2_PLACEMENT_3D('',#228506,#132779,#132780);
#107408=AXIS2_PLACEMENT_3D('',#228507,#132781,#132782);
#107409=AXIS2_PLACEMENT_3D('',#228510,#132783,#132784);
#107410=AXIS2_PLACEMENT_3D('',#228518,#132788,#132789);
#107411=AXIS2_PLACEMENT_3D('',#228524,#132792,#132793);
#107412=AXIS2_PLACEMENT_3D('',#228528,#132795,#132796);
#107413=AXIS2_PLACEMENT_3D('',#228532,#132799,#132800);
#107414=AXIS2_PLACEMENT_3D('',#228535,#132801,#132802);
#107415=AXIS2_PLACEMENT_3D('',#228543,#132806,#132807);
#107416=AXIS2_PLACEMENT_3D('',#228549,#132810,#132811);
#107417=AXIS2_PLACEMENT_3D('',#228553,#132813,#132814);
#107418=AXIS2_PLACEMENT_3D('',#228557,#132817,#132818);
#107419=AXIS2_PLACEMENT_3D('',#228562,#132820,#132821);
#107420=AXIS2_PLACEMENT_3D('',#228565,#132823,#132824);
#107421=AXIS2_PLACEMENT_3D('',#228566,#132825,#132826);
#107422=AXIS2_PLACEMENT_3D('',#228569,#132827,#132828);
#107423=AXIS2_PLACEMENT_3D('',#228577,#132832,#132833);
#107424=AXIS2_PLACEMENT_3D('',#228583,#132836,#132837);
#107425=AXIS2_PLACEMENT_3D('',#228587,#132839,#132840);
#107426=AXIS2_PLACEMENT_3D('',#228591,#132843,#132844);
#107427=AXIS2_PLACEMENT_3D('',#228594,#132845,#132846);
#107428=AXIS2_PLACEMENT_3D('',#228602,#132850,#132851);
#107429=AXIS2_PLACEMENT_3D('',#228608,#132854,#132855);
#107430=AXIS2_PLACEMENT_3D('',#228612,#132857,#132858);
#107431=AXIS2_PLACEMENT_3D('',#228616,#132861,#132862);
#107432=AXIS2_PLACEMENT_3D('',#228621,#132864,#132865);
#107433=AXIS2_PLACEMENT_3D('',#228624,#132867,#132868);
#107434=AXIS2_PLACEMENT_3D('',#228625,#132869,#132870);
#107435=AXIS2_PLACEMENT_3D('',#228628,#132871,#132872);
#107436=AXIS2_PLACEMENT_3D('',#228636,#132876,#132877);
#107437=AXIS2_PLACEMENT_3D('',#228642,#132880,#132881);
#107438=AXIS2_PLACEMENT_3D('',#228646,#132883,#132884);
#107439=AXIS2_PLACEMENT_3D('',#228650,#132887,#132888);
#107440=AXIS2_PLACEMENT_3D('',#228653,#132889,#132890);
#107441=AXIS2_PLACEMENT_3D('',#228661,#132894,#132895);
#107442=AXIS2_PLACEMENT_3D('',#228667,#132898,#132899);
#107443=AXIS2_PLACEMENT_3D('',#228671,#132901,#132902);
#107444=AXIS2_PLACEMENT_3D('',#228675,#132905,#132906);
#107445=AXIS2_PLACEMENT_3D('',#228680,#132908,#132909);
#107446=AXIS2_PLACEMENT_3D('',#228683,#132911,#132912);
#107447=AXIS2_PLACEMENT_3D('',#228684,#132913,#132914);
#107448=AXIS2_PLACEMENT_3D('',#228687,#132915,#132916);
#107449=AXIS2_PLACEMENT_3D('',#228695,#132920,#132921);
#107450=AXIS2_PLACEMENT_3D('',#228701,#132924,#132925);
#107451=AXIS2_PLACEMENT_3D('',#228705,#132927,#132928);
#107452=AXIS2_PLACEMENT_3D('',#228709,#132931,#132932);
#107453=AXIS2_PLACEMENT_3D('',#228712,#132933,#132934);
#107454=AXIS2_PLACEMENT_3D('',#228720,#132938,#132939);
#107455=AXIS2_PLACEMENT_3D('',#228726,#132942,#132943);
#107456=AXIS2_PLACEMENT_3D('',#228730,#132945,#132946);
#107457=AXIS2_PLACEMENT_3D('',#228734,#132949,#132950);
#107458=AXIS2_PLACEMENT_3D('',#228739,#132952,#132953);
#107459=AXIS2_PLACEMENT_3D('',#228742,#132955,#132956);
#107460=AXIS2_PLACEMENT_3D('',#228743,#132957,#132958);
#107461=AXIS2_PLACEMENT_3D('',#228746,#132959,#132960);
#107462=AXIS2_PLACEMENT_3D('',#228754,#132964,#132965);
#107463=AXIS2_PLACEMENT_3D('',#228760,#132968,#132969);
#107464=AXIS2_PLACEMENT_3D('',#228764,#132971,#132972);
#107465=AXIS2_PLACEMENT_3D('',#228768,#132975,#132976);
#107466=AXIS2_PLACEMENT_3D('',#228771,#132977,#132978);
#107467=AXIS2_PLACEMENT_3D('',#228779,#132982,#132983);
#107468=AXIS2_PLACEMENT_3D('',#228785,#132986,#132987);
#107469=AXIS2_PLACEMENT_3D('',#228789,#132989,#132990);
#107470=AXIS2_PLACEMENT_3D('',#228793,#132993,#132994);
#107471=AXIS2_PLACEMENT_3D('',#228798,#132996,#132997);
#107472=AXIS2_PLACEMENT_3D('',#228801,#132999,#133000);
#107473=AXIS2_PLACEMENT_3D('',#228802,#133001,#133002);
#107474=AXIS2_PLACEMENT_3D('',#228805,#133003,#133004);
#107475=AXIS2_PLACEMENT_3D('',#228813,#133008,#133009);
#107476=AXIS2_PLACEMENT_3D('',#228819,#133012,#133013);
#107477=AXIS2_PLACEMENT_3D('',#228823,#133015,#133016);
#107478=AXIS2_PLACEMENT_3D('',#228827,#133019,#133020);
#107479=AXIS2_PLACEMENT_3D('',#228830,#133021,#133022);
#107480=AXIS2_PLACEMENT_3D('',#228838,#133026,#133027);
#107481=AXIS2_PLACEMENT_3D('',#228844,#133030,#133031);
#107482=AXIS2_PLACEMENT_3D('',#228848,#133033,#133034);
#107483=AXIS2_PLACEMENT_3D('',#228852,#133037,#133038);
#107484=AXIS2_PLACEMENT_3D('',#228957,#133039,#133040);
#107485=AXIS2_PLACEMENT_3D('',#229056,#133041,#133042);
#107486=AXIS2_PLACEMENT_3D('',#229161,#133043,#133044);
#107487=AXIS2_PLACEMENT_3D('',#229260,#133045,#133046);
#107488=AXIS2_PLACEMENT_3D('',#229365,#133047,#133048);
#107489=AXIS2_PLACEMENT_3D('',#229464,#133049,#133050);
#107490=AXIS2_PLACEMENT_3D('',#229569,#133051,#133052);
#107491=AXIS2_PLACEMENT_3D('',#229668,#133053,#133054);
#107492=AXIS2_PLACEMENT_3D('',#229773,#133055,#133056);
#107493=AXIS2_PLACEMENT_3D('',#229872,#133057,#133058);
#107494=AXIS2_PLACEMENT_3D('',#229977,#133059,#133060);
#107495=AXIS2_PLACEMENT_3D('',#230076,#133061,#133062);
#107496=AXIS2_PLACEMENT_3D('',#230181,#133063,#133064);
#107497=AXIS2_PLACEMENT_3D('',#230280,#133065,#133066);
#107498=AXIS2_PLACEMENT_3D('',#230385,#133067,#133068);
#107499=AXIS2_PLACEMENT_3D('',#230484,#133069,#133070);
#107500=AXIS2_PLACEMENT_3D('',#230589,#133071,#133072);
#107501=AXIS2_PLACEMENT_3D('',#230688,#133073,#133074);
#107502=AXIS2_PLACEMENT_3D('',#230793,#133075,#133076);
#107503=AXIS2_PLACEMENT_3D('',#230892,#133077,#133078);
#107504=AXIS2_PLACEMENT_3D('',#230997,#133079,#133080);
#107505=AXIS2_PLACEMENT_3D('',#231096,#133081,#133082);
#107506=AXIS2_PLACEMENT_3D('',#231201,#133083,#133084);
#107507=AXIS2_PLACEMENT_3D('',#231300,#133085,#133086);
#107508=AXIS2_PLACEMENT_3D('',#231405,#133087,#133088);
#107509=AXIS2_PLACEMENT_3D('',#231504,#133089,#133090);
#107510=AXIS2_PLACEMENT_3D('',#231609,#133091,#133092);
#107511=AXIS2_PLACEMENT_3D('',#231708,#133093,#133094);
#107512=AXIS2_PLACEMENT_3D('',#231813,#133095,#133096);
#107513=AXIS2_PLACEMENT_3D('',#231912,#133097,#133098);
#107514=AXIS2_PLACEMENT_3D('',#232017,#133099,#133100);
#107515=AXIS2_PLACEMENT_3D('',#232116,#133101,#133102);
#107516=AXIS2_PLACEMENT_3D('',#232221,#133103,#133104);
#107517=AXIS2_PLACEMENT_3D('',#232320,#133105,#133106);
#107518=AXIS2_PLACEMENT_3D('',#232425,#133107,#133108);
#107519=AXIS2_PLACEMENT_3D('',#232524,#133109,#133110);
#107520=AXIS2_PLACEMENT_3D('',#232629,#133111,#133112);
#107521=AXIS2_PLACEMENT_3D('',#232728,#133113,#133114);
#107522=AXIS2_PLACEMENT_3D('',#232833,#133115,#133116);
#107523=AXIS2_PLACEMENT_3D('',#232932,#133117,#133118);
#107524=AXIS2_PLACEMENT_3D('',#233037,#133119,#133120);
#107525=AXIS2_PLACEMENT_3D('',#233136,#133121,#133122);
#107526=AXIS2_PLACEMENT_3D('',#233241,#133123,#133124);
#107527=AXIS2_PLACEMENT_3D('',#233340,#133125,#133126);
#107528=AXIS2_PLACEMENT_3D('',#233445,#133127,#133128);
#107529=AXIS2_PLACEMENT_3D('',#233544,#133129,#133130);
#107530=AXIS2_PLACEMENT_3D('',#233649,#133131,#133132);
#107531=AXIS2_PLACEMENT_3D('',#233748,#133133,#133134);
#107532=AXIS2_PLACEMENT_3D('',#233853,#133135,#133136);
#107533=AXIS2_PLACEMENT_3D('',#233952,#133137,#133138);
#107534=AXIS2_PLACEMENT_3D('',#234057,#133139,#133140);
#107535=AXIS2_PLACEMENT_3D('',#234156,#133141,#133142);
#107536=AXIS2_PLACEMENT_3D('',#234261,#133143,#133144);
#107537=AXIS2_PLACEMENT_3D('',#234360,#133145,#133146);
#107538=AXIS2_PLACEMENT_3D('',#234465,#133147,#133148);
#107539=AXIS2_PLACEMENT_3D('',#234564,#133149,#133150);
#107540=AXIS2_PLACEMENT_3D('',#234669,#133151,#133152);
#107541=AXIS2_PLACEMENT_3D('',#234768,#133153,#133154);
#107542=AXIS2_PLACEMENT_3D('',#234873,#133155,#133156);
#107543=AXIS2_PLACEMENT_3D('',#234972,#133157,#133158);
#107544=AXIS2_PLACEMENT_3D('',#235077,#133159,#133160);
#107545=AXIS2_PLACEMENT_3D('',#235176,#133161,#133162);
#107546=AXIS2_PLACEMENT_3D('',#235281,#133163,#133164);
#107547=AXIS2_PLACEMENT_3D('',#235380,#133165,#133166);
#107548=AXIS2_PLACEMENT_3D('',#235485,#133167,#133168);
#107549=AXIS2_PLACEMENT_3D('',#235584,#133169,#133170);
#107550=AXIS2_PLACEMENT_3D('',#235689,#133171,#133172);
#107551=AXIS2_PLACEMENT_3D('',#235788,#133173,#133174);
#107552=AXIS2_PLACEMENT_3D('',#235893,#133175,#133176);
#107553=AXIS2_PLACEMENT_3D('',#235992,#133177,#133178);
#107554=AXIS2_PLACEMENT_3D('',#236097,#133179,#133180);
#107555=AXIS2_PLACEMENT_3D('',#236196,#133181,#133182);
#107556=AXIS2_PLACEMENT_3D('',#236301,#133183,#133184);
#107557=AXIS2_PLACEMENT_3D('',#236400,#133185,#133186);
#107558=AXIS2_PLACEMENT_3D('',#236505,#133187,#133188);
#107559=AXIS2_PLACEMENT_3D('',#236604,#133189,#133190);
#107560=AXIS2_PLACEMENT_3D('',#236709,#133191,#133192);
#107561=AXIS2_PLACEMENT_3D('',#236808,#133193,#133194);
#107562=AXIS2_PLACEMENT_3D('',#236913,#133195,#133196);
#107563=AXIS2_PLACEMENT_3D('',#237012,#133197,#133198);
#107564=AXIS2_PLACEMENT_3D('',#237117,#133199,#133200);
#107565=AXIS2_PLACEMENT_3D('',#237216,#133201,#133202);
#107566=AXIS2_PLACEMENT_3D('',#237321,#133203,#133204);
#107567=AXIS2_PLACEMENT_3D('',#237420,#133205,#133206);
#107568=AXIS2_PLACEMENT_3D('',#237525,#133207,#133208);
#107569=AXIS2_PLACEMENT_3D('',#237624,#133209,#133210);
#107570=AXIS2_PLACEMENT_3D('',#237729,#133211,#133212);
#107571=AXIS2_PLACEMENT_3D('',#237828,#133213,#133214);
#107572=AXIS2_PLACEMENT_3D('',#237933,#133215,#133216);
#107573=AXIS2_PLACEMENT_3D('',#238032,#133217,#133218);
#107574=AXIS2_PLACEMENT_3D('',#238137,#133219,#133220);
#107575=AXIS2_PLACEMENT_3D('',#238236,#133221,#133222);
#107576=AXIS2_PLACEMENT_3D('',#238341,#133223,#133224);
#107577=AXIS2_PLACEMENT_3D('',#238440,#133225,#133226);
#107578=AXIS2_PLACEMENT_3D('',#238545,#133227,#133228);
#107579=AXIS2_PLACEMENT_3D('',#238644,#133229,#133230);
#107580=AXIS2_PLACEMENT_3D('',#238749,#133231,#133232);
#107581=AXIS2_PLACEMENT_3D('',#238848,#133233,#133234);
#107582=AXIS2_PLACEMENT_3D('',#238953,#133235,#133236);
#107583=AXIS2_PLACEMENT_3D('',#239052,#133237,#133238);
#107584=AXIS2_PLACEMENT_3D('',#239157,#133239,#133240);
#107585=AXIS2_PLACEMENT_3D('',#239256,#133241,#133242);
#107586=AXIS2_PLACEMENT_3D('',#239361,#133243,#133244);
#107587=AXIS2_PLACEMENT_3D('',#239460,#133245,#133246);
#107588=AXIS2_PLACEMENT_3D('',#239565,#133247,#133248);
#107589=AXIS2_PLACEMENT_3D('',#239664,#133249,#133250);
#107590=AXIS2_PLACEMENT_3D('',#239769,#133251,#133252);
#107591=AXIS2_PLACEMENT_3D('',#239868,#133253,#133254);
#107592=AXIS2_PLACEMENT_3D('',#239973,#133255,#133256);
#107593=AXIS2_PLACEMENT_3D('',#240072,#133257,#133258);
#107594=AXIS2_PLACEMENT_3D('',#240177,#133259,#133260);
#107595=AXIS2_PLACEMENT_3D('',#240276,#133261,#133262);
#107596=AXIS2_PLACEMENT_3D('',#240381,#133263,#133264);
#107597=AXIS2_PLACEMENT_3D('',#240480,#133265,#133266);
#107598=AXIS2_PLACEMENT_3D('',#240585,#133267,#133268);
#107599=AXIS2_PLACEMENT_3D('',#240684,#133269,#133270);
#107600=AXIS2_PLACEMENT_3D('',#240789,#133271,#133272);
#107601=AXIS2_PLACEMENT_3D('',#240888,#133273,#133274);
#107602=AXIS2_PLACEMENT_3D('',#240889,#133275,#133276);
#107603=AXIS2_PLACEMENT_3D('',#240890,#133277,#133278);
#107604=AXIS2_PLACEMENT_3D('',#240903,#133279,#133280);
#107605=AXIS2_PLACEMENT_3D('',#240904,#133281,#133282);
#107606=AXIS2_PLACEMENT_3D('',#240905,#133283,#133284);
#107607=AXIS2_PLACEMENT_3D('',#240906,#133285,#133286);
#107608=AXIS2_PLACEMENT_3D('',#240907,#133287,#133288);
#107609=AXIS2_PLACEMENT_3D('',#240920,#133289,#133290);
#107610=AXIS2_PLACEMENT_3D('',#240933,#133291,#133292);
#107611=AXIS2_PLACEMENT_3D('',#240934,#133293,#133294);
#107612=AXIS2_PLACEMENT_3D('',#240935,#133295,#133296);
#107613=AXIS2_PLACEMENT_3D('',#240936,#133297,#133298);
#107614=AXIS2_PLACEMENT_3D('',#240937,#133299,#133300);
#107615=AXIS2_PLACEMENT_3D('',#240956,#133301,#133302);
#107616=AXIS2_PLACEMENT_3D('',#240957,#133303,#133304);
#107617=AXIS2_PLACEMENT_3D('',#240958,#133305,#133306);
#107618=AXIS2_PLACEMENT_3D('',#240959,#133307,#133308);
#107619=AXIS2_PLACEMENT_3D('',#240960,#133309,#133310);
#107620=AXIS2_PLACEMENT_3D('',#240973,#133311,#133312);
#107621=AXIS2_PLACEMENT_3D('',#240992,#133313,#133314);
#107622=AXIS2_PLACEMENT_3D('',#240993,#133315,#133316);
#107623=AXIS2_PLACEMENT_3D('',#240994,#133317,#133318);
#107624=AXIS2_PLACEMENT_3D('',#240995,#133319,#133320);
#107625=AXIS2_PLACEMENT_3D('',#240996,#133321,#133322);
#107626=AXIS2_PLACEMENT_3D('',#241015,#133323,#133324);
#107627=AXIS2_PLACEMENT_3D('',#241028,#133325,#133326);
#107628=AXIS2_PLACEMENT_3D('',#241029,#133327,#133328);
#107629=AXIS2_PLACEMENT_3D('',#241030,#133329,#133330);
#107630=AXIS2_PLACEMENT_3D('',#241031,#133331,#133332);
#107631=AXIS2_PLACEMENT_3D('',#241032,#133333,#133334);
#107632=AXIS2_PLACEMENT_3D('',#241051,#133335,#133336);
#107633=AXIS2_PLACEMENT_3D('',#241052,#133337,#133338);
#107634=AXIS2_PLACEMENT_3D('',#241053,#133339,#133340);
#107635=AXIS2_PLACEMENT_3D('',#241054,#133341,#133342);
#107636=AXIS2_PLACEMENT_3D('',#241055,#133343,#133344);
#107637=AXIS2_PLACEMENT_3D('',#241068,#133345,#133346);
#107638=AXIS2_PLACEMENT_3D('',#241081,#133347,#133348);
#107639=AXIS2_PLACEMENT_3D('',#241082,#133349,#133350);
#107640=AXIS2_PLACEMENT_3D('',#241083,#133351,#133352);
#107641=AXIS2_PLACEMENT_3D('',#241084,#133353,#133354);
#107642=AXIS2_PLACEMENT_3D('',#241085,#133355,#133356);
#107643=AXIS2_PLACEMENT_3D('',#241098,#133357,#133358);
#107644=AXIS2_PLACEMENT_3D('',#241099,#133359,#133360);
#107645=AXIS2_PLACEMENT_3D('',#241100,#133361,#133362);
#107646=AXIS2_PLACEMENT_3D('',#241101,#133363,#133364);
#107647=AXIS2_PLACEMENT_3D('',#241102,#133365,#133366);
#107648=AXIS2_PLACEMENT_3D('',#241115,#133367,#133368);
#107649=AXIS2_PLACEMENT_3D('',#241116,#133369,#133370);
#107650=AXIS2_PLACEMENT_3D('',#241117,#133371,#133372);
#107651=AXIS2_PLACEMENT_3D('',#241118,#133373,#133374);
#107652=AXIS2_PLACEMENT_3D('',#241119,#133375,#133376);
#107653=AXIS2_PLACEMENT_3D('',#241132,#133377,#133378);
#107654=AXIS2_PLACEMENT_3D('',#241145,#133379,#133380);
#107655=AXIS2_PLACEMENT_3D('',#241146,#133381,#133382);
#107656=AXIS2_PLACEMENT_3D('',#241147,#133383,#133384);
#107657=AXIS2_PLACEMENT_3D('',#241148,#133385,#133386);
#107658=AXIS2_PLACEMENT_3D('',#241149,#133387,#133388);
#107659=AXIS2_PLACEMENT_3D('',#241168,#133389,#133390);
#107660=AXIS2_PLACEMENT_3D('',#241169,#133391,#133392);
#107661=AXIS2_PLACEMENT_3D('',#241170,#133393,#133394);
#107662=AXIS2_PLACEMENT_3D('',#241171,#133395,#133396);
#107663=AXIS2_PLACEMENT_3D('',#241172,#133397,#133398);
#107664=AXIS2_PLACEMENT_3D('',#241185,#133399,#133400);
#107665=AXIS2_PLACEMENT_3D('',#241204,#133401,#133402);
#107666=AXIS2_PLACEMENT_3D('',#241205,#133403,#133404);
#107667=AXIS2_PLACEMENT_3D('',#241206,#133405,#133406);
#107668=AXIS2_PLACEMENT_3D('',#241207,#133407,#133408);
#107669=AXIS2_PLACEMENT_3D('',#241208,#133409,#133410);
#107670=AXIS2_PLACEMENT_3D('',#241227,#133411,#133412);
#107671=AXIS2_PLACEMENT_3D('',#241240,#133413,#133414);
#107672=AXIS2_PLACEMENT_3D('',#241241,#133415,#133416);
#107673=AXIS2_PLACEMENT_3D('',#241242,#133417,#133418);
#107674=AXIS2_PLACEMENT_3D('',#241243,#133419,#133420);
#107675=AXIS2_PLACEMENT_3D('',#241244,#133421,#133422);
#107676=AXIS2_PLACEMENT_3D('',#241263,#133423,#133424);
#107677=AXIS2_PLACEMENT_3D('',#241264,#133425,#133426);
#107678=AXIS2_PLACEMENT_3D('',#241265,#133427,#133428);
#107679=AXIS2_PLACEMENT_3D('',#241266,#133429,#133430);
#107680=AXIS2_PLACEMENT_3D('',#241267,#133431,#133432);
#107681=AXIS2_PLACEMENT_3D('',#241280,#133433,#133434);
#107682=AXIS2_PLACEMENT_3D('',#241293,#133435,#133436);
#107683=AXIS2_PLACEMENT_3D('',#241294,#133437,#133438);
#107684=AXIS2_PLACEMENT_3D('',#241295,#133439,#133440);
#107685=AXIS2_PLACEMENT_3D('',#241296,#133441,#133442);
#107686=AXIS2_PLACEMENT_3D('',#241297,#133443,#133444);
#107687=AXIS2_PLACEMENT_3D('',#241310,#133445,#133446);
#107688=AXIS2_PLACEMENT_3D('',#241311,#133447,#133448);
#107689=AXIS2_PLACEMENT_3D('',#241312,#133449,#133450);
#107690=AXIS2_PLACEMENT_3D('',#241313,#133451,#133452);
#107691=AXIS2_PLACEMENT_3D('',#241314,#133453,#133454);
#107692=AXIS2_PLACEMENT_3D('',#241327,#133455,#133456);
#107693=AXIS2_PLACEMENT_3D('',#241328,#133457,#133458);
#107694=AXIS2_PLACEMENT_3D('',#241329,#133459,#133460);
#107695=AXIS2_PLACEMENT_3D('',#241330,#133461,#133462);
#107696=AXIS2_PLACEMENT_3D('',#241331,#133463,#133464);
#107697=AXIS2_PLACEMENT_3D('',#241344,#133465,#133466);
#107698=AXIS2_PLACEMENT_3D('',#241357,#133467,#133468);
#107699=AXIS2_PLACEMENT_3D('',#241358,#133469,#133470);
#107700=AXIS2_PLACEMENT_3D('',#241359,#133471,#133472);
#107701=AXIS2_PLACEMENT_3D('',#241360,#133473,#133474);
#107702=AXIS2_PLACEMENT_3D('',#241361,#133475,#133476);
#107703=AXIS2_PLACEMENT_3D('',#241380,#133477,#133478);
#107704=AXIS2_PLACEMENT_3D('',#241381,#133479,#133480);
#107705=AXIS2_PLACEMENT_3D('',#241382,#133481,#133482);
#107706=AXIS2_PLACEMENT_3D('',#241383,#133483,#133484);
#107707=AXIS2_PLACEMENT_3D('',#241384,#133485,#133486);
#107708=AXIS2_PLACEMENT_3D('',#241397,#133487,#133488);
#107709=AXIS2_PLACEMENT_3D('',#241416,#133489,#133490);
#107710=AXIS2_PLACEMENT_3D('',#241417,#133491,#133492);
#107711=AXIS2_PLACEMENT_3D('',#241418,#133493,#133494);
#107712=AXIS2_PLACEMENT_3D('',#241419,#133495,#133496);
#107713=AXIS2_PLACEMENT_3D('',#241420,#133497,#133498);
#107714=AXIS2_PLACEMENT_3D('',#241439,#133499,#133500);
#107715=AXIS2_PLACEMENT_3D('',#241452,#133501,#133502);
#107716=AXIS2_PLACEMENT_3D('',#241453,#133503,#133504);
#107717=AXIS2_PLACEMENT_3D('',#241454,#133505,#133506);
#107718=AXIS2_PLACEMENT_3D('',#241455,#133507,#133508);
#107719=AXIS2_PLACEMENT_3D('',#241456,#133509,#133510);
#107720=AXIS2_PLACEMENT_3D('',#241475,#133511,#133512);
#107721=AXIS2_PLACEMENT_3D('',#241476,#133513,#133514);
#107722=AXIS2_PLACEMENT_3D('',#241477,#133515,#133516);
#107723=AXIS2_PLACEMENT_3D('',#241478,#133517,#133518);
#107724=AXIS2_PLACEMENT_3D('',#241479,#133519,#133520);
#107725=AXIS2_PLACEMENT_3D('',#241492,#133521,#133522);
#107726=AXIS2_PLACEMENT_3D('',#241505,#133523,#133524);
#107727=AXIS2_PLACEMENT_3D('',#241506,#133525,#133526);
#107728=AXIS2_PLACEMENT_3D('',#241507,#133527,#133528);
#107729=AXIS2_PLACEMENT_3D('',#241508,#133529,#133530);
#107730=AXIS2_PLACEMENT_3D('',#241509,#133531,#133532);
#107731=AXIS2_PLACEMENT_3D('',#241522,#133533,#133534);
#107732=AXIS2_PLACEMENT_3D('',#241523,#133535,#133536);
#107733=AXIS2_PLACEMENT_3D('',#241524,#133537,#133538);
#107734=AXIS2_PLACEMENT_3D('',#241525,#133539,#133540);
#107735=AXIS2_PLACEMENT_3D('',#241526,#133541,#133542);
#107736=AXIS2_PLACEMENT_3D('',#241539,#133543,#133544);
#107737=AXIS2_PLACEMENT_3D('',#241540,#133545,#133546);
#107738=AXIS2_PLACEMENT_3D('',#241541,#133547,#133548);
#107739=AXIS2_PLACEMENT_3D('',#241542,#133549,#133550);
#107740=AXIS2_PLACEMENT_3D('',#241543,#133551,#133552);
#107741=AXIS2_PLACEMENT_3D('',#241556,#133553,#133554);
#107742=AXIS2_PLACEMENT_3D('',#241569,#133555,#133556);
#107743=AXIS2_PLACEMENT_3D('',#241570,#133557,#133558);
#107744=AXIS2_PLACEMENT_3D('',#241571,#133559,#133560);
#107745=AXIS2_PLACEMENT_3D('',#241572,#133561,#133562);
#107746=AXIS2_PLACEMENT_3D('',#241573,#133563,#133564);
#107747=AXIS2_PLACEMENT_3D('',#241592,#133565,#133566);
#107748=AXIS2_PLACEMENT_3D('',#241593,#133567,#133568);
#107749=AXIS2_PLACEMENT_3D('',#241594,#133569,#133570);
#107750=AXIS2_PLACEMENT_3D('',#241595,#133571,#133572);
#107751=AXIS2_PLACEMENT_3D('',#241596,#133573,#133574);
#107752=AXIS2_PLACEMENT_3D('',#241609,#133575,#133576);
#107753=AXIS2_PLACEMENT_3D('',#241628,#133577,#133578);
#107754=AXIS2_PLACEMENT_3D('',#241629,#133579,#133580);
#107755=AXIS2_PLACEMENT_3D('',#241630,#133581,#133582);
#107756=AXIS2_PLACEMENT_3D('',#241631,#133583,#133584);
#107757=AXIS2_PLACEMENT_3D('',#241632,#133585,#133586);
#107758=AXIS2_PLACEMENT_3D('',#241651,#133587,#133588);
#107759=AXIS2_PLACEMENT_3D('',#241664,#133589,#133590);
#107760=AXIS2_PLACEMENT_3D('',#241665,#133591,#133592);
#107761=AXIS2_PLACEMENT_3D('',#241666,#133593,#133594);
#107762=AXIS2_PLACEMENT_3D('',#241667,#133595,#133596);
#107763=AXIS2_PLACEMENT_3D('',#241668,#133597,#133598);
#107764=AXIS2_PLACEMENT_3D('',#241687,#133599,#133600);
#107765=AXIS2_PLACEMENT_3D('',#241688,#133601,#133602);
#107766=AXIS2_PLACEMENT_3D('',#241689,#133603,#133604);
#107767=AXIS2_PLACEMENT_3D('',#241690,#133605,#133606);
#107768=AXIS2_PLACEMENT_3D('',#241691,#133607,#133608);
#107769=AXIS2_PLACEMENT_3D('',#241704,#133609,#133610);
#107770=AXIS2_PLACEMENT_3D('',#241717,#133611,#133612);
#107771=AXIS2_PLACEMENT_3D('',#241718,#133613,#133614);
#107772=AXIS2_PLACEMENT_3D('',#241719,#133615,#133616);
#107773=AXIS2_PLACEMENT_3D('',#241720,#133617,#133618);
#107774=AXIS2_PLACEMENT_3D('',#241721,#133619,#133620);
#107775=AXIS2_PLACEMENT_3D('',#241734,#133621,#133622);
#107776=AXIS2_PLACEMENT_3D('',#241735,#133623,#133624);
#107777=AXIS2_PLACEMENT_3D('',#241736,#133625,#133626);
#107778=AXIS2_PLACEMENT_3D('',#241737,#133627,#133628);
#107779=AXIS2_PLACEMENT_3D('',#241738,#133629,#133630);
#107780=AXIS2_PLACEMENT_3D('',#241751,#133631,#133632);
#107781=AXIS2_PLACEMENT_3D('',#241752,#133633,#133634);
#107782=AXIS2_PLACEMENT_3D('',#241753,#133635,#133636);
#107783=AXIS2_PLACEMENT_3D('',#241754,#133637,#133638);
#107784=AXIS2_PLACEMENT_3D('',#241755,#133639,#133640);
#107785=AXIS2_PLACEMENT_3D('',#241768,#133641,#133642);
#107786=AXIS2_PLACEMENT_3D('',#241781,#133643,#133644);
#107787=AXIS2_PLACEMENT_3D('',#241782,#133645,#133646);
#107788=AXIS2_PLACEMENT_3D('',#241783,#133647,#133648);
#107789=AXIS2_PLACEMENT_3D('',#241784,#133649,#133650);
#107790=AXIS2_PLACEMENT_3D('',#241785,#133651,#133652);
#107791=AXIS2_PLACEMENT_3D('',#241804,#133653,#133654);
#107792=AXIS2_PLACEMENT_3D('',#241805,#133655,#133656);
#107793=AXIS2_PLACEMENT_3D('',#241806,#133657,#133658);
#107794=AXIS2_PLACEMENT_3D('',#241807,#133659,#133660);
#107795=AXIS2_PLACEMENT_3D('',#241808,#133661,#133662);
#107796=AXIS2_PLACEMENT_3D('',#241821,#133663,#133664);
#107797=AXIS2_PLACEMENT_3D('',#241840,#133665,#133666);
#107798=AXIS2_PLACEMENT_3D('',#241841,#133667,#133668);
#107799=AXIS2_PLACEMENT_3D('',#241842,#133669,#133670);
#107800=AXIS2_PLACEMENT_3D('',#241843,#133671,#133672);
#107801=AXIS2_PLACEMENT_3D('',#241844,#133673,#133674);
#107802=AXIS2_PLACEMENT_3D('',#241863,#133675,#133676);
#107803=AXIS2_PLACEMENT_3D('',#241876,#133677,#133678);
#107804=AXIS2_PLACEMENT_3D('',#241877,#133679,#133680);
#107805=AXIS2_PLACEMENT_3D('',#241878,#133681,#133682);
#107806=AXIS2_PLACEMENT_3D('',#241879,#133683,#133684);
#107807=AXIS2_PLACEMENT_3D('',#241880,#133685,#133686);
#107808=AXIS2_PLACEMENT_3D('',#241899,#133687,#133688);
#107809=AXIS2_PLACEMENT_3D('',#241900,#133689,#133690);
#107810=AXIS2_PLACEMENT_3D('',#241901,#133691,#133692);
#107811=AXIS2_PLACEMENT_3D('',#241902,#133693,#133694);
#107812=AXIS2_PLACEMENT_3D('',#241903,#133695,#133696);
#107813=AXIS2_PLACEMENT_3D('',#241916,#133697,#133698);
#107814=AXIS2_PLACEMENT_3D('',#241929,#133699,#133700);
#107815=AXIS2_PLACEMENT_3D('',#241930,#133701,#133702);
#107816=AXIS2_PLACEMENT_3D('',#241931,#133703,#133704);
#107817=AXIS2_PLACEMENT_3D('',#241932,#133705,#133706);
#107818=AXIS2_PLACEMENT_3D('',#241933,#133707,#133708);
#107819=AXIS2_PLACEMENT_3D('',#241946,#133709,#133710);
#107820=AXIS2_PLACEMENT_3D('',#241947,#133711,#133712);
#107821=AXIS2_PLACEMENT_3D('',#241948,#133713,#133714);
#107822=AXIS2_PLACEMENT_3D('',#241949,#133715,#133716);
#107823=AXIS2_PLACEMENT_3D('',#241950,#133717,#133718);
#107824=AXIS2_PLACEMENT_3D('',#241963,#133719,#133720);
#107825=AXIS2_PLACEMENT_3D('',#241964,#133721,#133722);
#107826=AXIS2_PLACEMENT_3D('',#241965,#133723,#133724);
#107827=AXIS2_PLACEMENT_3D('',#241966,#133725,#133726);
#107828=AXIS2_PLACEMENT_3D('',#241967,#133727,#133728);
#107829=AXIS2_PLACEMENT_3D('',#241980,#133729,#133730);
#107830=AXIS2_PLACEMENT_3D('',#241993,#133731,#133732);
#107831=AXIS2_PLACEMENT_3D('',#241994,#133733,#133734);
#107832=AXIS2_PLACEMENT_3D('',#241995,#133735,#133736);
#107833=AXIS2_PLACEMENT_3D('',#241996,#133737,#133738);
#107834=AXIS2_PLACEMENT_3D('',#241997,#133739,#133740);
#107835=AXIS2_PLACEMENT_3D('',#242016,#133741,#133742);
#107836=AXIS2_PLACEMENT_3D('',#242017,#133743,#133744);
#107837=AXIS2_PLACEMENT_3D('',#242018,#133745,#133746);
#107838=AXIS2_PLACEMENT_3D('',#242019,#133747,#133748);
#107839=AXIS2_PLACEMENT_3D('',#242020,#133749,#133750);
#107840=AXIS2_PLACEMENT_3D('',#242033,#133751,#133752);
#107841=AXIS2_PLACEMENT_3D('',#242052,#133753,#133754);
#107842=AXIS2_PLACEMENT_3D('',#242053,#133755,#133756);
#107843=AXIS2_PLACEMENT_3D('',#242054,#133757,#133758);
#107844=AXIS2_PLACEMENT_3D('',#242055,#133759,#133760);
#107845=AXIS2_PLACEMENT_3D('',#242056,#133761,#133762);
#107846=AXIS2_PLACEMENT_3D('',#242075,#133763,#133764);
#107847=AXIS2_PLACEMENT_3D('',#242088,#133765,#133766);
#107848=AXIS2_PLACEMENT_3D('',#242089,#133767,#133768);
#107849=AXIS2_PLACEMENT_3D('',#242090,#133769,#133770);
#107850=AXIS2_PLACEMENT_3D('',#242091,#133771,#133772);
#107851=AXIS2_PLACEMENT_3D('',#242092,#133773,#133774);
#107852=AXIS2_PLACEMENT_3D('',#242111,#133775,#133776);
#107853=AXIS2_PLACEMENT_3D('',#242112,#133777,#133778);
#107854=AXIS2_PLACEMENT_3D('',#242113,#133779,#133780);
#107855=AXIS2_PLACEMENT_3D('',#242114,#133781,#133782);
#107856=AXIS2_PLACEMENT_3D('',#242115,#133783,#133784);
#107857=AXIS2_PLACEMENT_3D('',#242128,#133785,#133786);
#107858=AXIS2_PLACEMENT_3D('',#242141,#133787,#133788);
#107859=AXIS2_PLACEMENT_3D('',#242142,#133789,#133790);
#107860=AXIS2_PLACEMENT_3D('',#242143,#133791,#133792);
#107861=AXIS2_PLACEMENT_3D('',#242144,#133793,#133794);
#107862=AXIS2_PLACEMENT_3D('',#242145,#133795,#133796);
#107863=AXIS2_PLACEMENT_3D('',#242158,#133797,#133798);
#107864=AXIS2_PLACEMENT_3D('',#242159,#133799,#133800);
#107865=AXIS2_PLACEMENT_3D('',#242160,#133801,#133802);
#107866=AXIS2_PLACEMENT_3D('',#242161,#133803,#133804);
#107867=AXIS2_PLACEMENT_3D('',#242162,#133805,#133806);
#107868=AXIS2_PLACEMENT_3D('',#242175,#133807,#133808);
#107869=AXIS2_PLACEMENT_3D('',#242176,#133809,#133810);
#107870=AXIS2_PLACEMENT_3D('',#242177,#133811,#133812);
#107871=AXIS2_PLACEMENT_3D('',#242178,#133813,#133814);
#107872=AXIS2_PLACEMENT_3D('',#242179,#133815,#133816);
#107873=AXIS2_PLACEMENT_3D('',#242192,#133817,#133818);
#107874=AXIS2_PLACEMENT_3D('',#242205,#133819,#133820);
#107875=AXIS2_PLACEMENT_3D('',#242206,#133821,#133822);
#107876=AXIS2_PLACEMENT_3D('',#242207,#133823,#133824);
#107877=AXIS2_PLACEMENT_3D('',#242208,#133825,#133826);
#107878=AXIS2_PLACEMENT_3D('',#242209,#133827,#133828);
#107879=AXIS2_PLACEMENT_3D('',#242228,#133829,#133830);
#107880=AXIS2_PLACEMENT_3D('',#242229,#133831,#133832);
#107881=AXIS2_PLACEMENT_3D('',#242230,#133833,#133834);
#107882=AXIS2_PLACEMENT_3D('',#242231,#133835,#133836);
#107883=AXIS2_PLACEMENT_3D('',#242232,#133837,#133838);
#107884=AXIS2_PLACEMENT_3D('',#242245,#133839,#133840);
#107885=AXIS2_PLACEMENT_3D('',#242264,#133841,#133842);
#107886=AXIS2_PLACEMENT_3D('',#242265,#133843,#133844);
#107887=AXIS2_PLACEMENT_3D('',#242266,#133845,#133846);
#107888=AXIS2_PLACEMENT_3D('',#242267,#133847,#133848);
#107889=AXIS2_PLACEMENT_3D('',#242268,#133849,#133850);
#107890=AXIS2_PLACEMENT_3D('',#242287,#133851,#133852);
#107891=AXIS2_PLACEMENT_3D('',#242300,#133853,#133854);
#107892=AXIS2_PLACEMENT_3D('',#242301,#133855,#133856);
#107893=AXIS2_PLACEMENT_3D('',#242302,#133857,#133858);
#107894=AXIS2_PLACEMENT_3D('',#242303,#133859,#133860);
#107895=AXIS2_PLACEMENT_3D('',#242304,#133861,#133862);
#107896=AXIS2_PLACEMENT_3D('',#242323,#133863,#133864);
#107897=AXIS2_PLACEMENT_3D('',#242324,#133865,#133866);
#107898=AXIS2_PLACEMENT_3D('',#242325,#133867,#133868);
#107899=AXIS2_PLACEMENT_3D('',#242326,#133869,#133870);
#107900=AXIS2_PLACEMENT_3D('',#242327,#133871,#133872);
#107901=AXIS2_PLACEMENT_3D('',#242340,#133873,#133874);
#107902=AXIS2_PLACEMENT_3D('',#242353,#133875,#133876);
#107903=AXIS2_PLACEMENT_3D('',#242354,#133877,#133878);
#107904=AXIS2_PLACEMENT_3D('',#242355,#133879,#133880);
#107905=AXIS2_PLACEMENT_3D('',#242356,#133881,#133882);
#107906=AXIS2_PLACEMENT_3D('',#242357,#133883,#133884);
#107907=AXIS2_PLACEMENT_3D('',#242370,#133885,#133886);
#107908=AXIS2_PLACEMENT_3D('',#242371,#133887,#133888);
#107909=AXIS2_PLACEMENT_3D('',#242372,#133889,#133890);
#107910=AXIS2_PLACEMENT_3D('',#242373,#133891,#133892);
#107911=AXIS2_PLACEMENT_3D('',#242374,#133893,#133894);
#107912=AXIS2_PLACEMENT_3D('',#242387,#133895,#133896);
#107913=AXIS2_PLACEMENT_3D('',#242388,#133897,#133898);
#107914=AXIS2_PLACEMENT_3D('',#242389,#133899,#133900);
#107915=AXIS2_PLACEMENT_3D('',#242390,#133901,#133902);
#107916=AXIS2_PLACEMENT_3D('',#242391,#133903,#133904);
#107917=AXIS2_PLACEMENT_3D('',#242404,#133905,#133906);
#107918=AXIS2_PLACEMENT_3D('',#242417,#133907,#133908);
#107919=AXIS2_PLACEMENT_3D('',#242418,#133909,#133910);
#107920=AXIS2_PLACEMENT_3D('',#242419,#133911,#133912);
#107921=AXIS2_PLACEMENT_3D('',#242420,#133913,#133914);
#107922=AXIS2_PLACEMENT_3D('',#242421,#133915,#133916);
#107923=AXIS2_PLACEMENT_3D('',#242440,#133917,#133918);
#107924=AXIS2_PLACEMENT_3D('',#242441,#133919,#133920);
#107925=AXIS2_PLACEMENT_3D('',#242442,#133921,#133922);
#107926=AXIS2_PLACEMENT_3D('',#242443,#133923,#133924);
#107927=AXIS2_PLACEMENT_3D('',#242444,#133925,#133926);
#107928=AXIS2_PLACEMENT_3D('',#242457,#133927,#133928);
#107929=AXIS2_PLACEMENT_3D('',#242476,#133929,#133930);
#107930=AXIS2_PLACEMENT_3D('',#242477,#133931,#133932);
#107931=AXIS2_PLACEMENT_3D('',#242478,#133933,#133934);
#107932=AXIS2_PLACEMENT_3D('',#242479,#133935,#133936);
#107933=AXIS2_PLACEMENT_3D('',#242480,#133937,#133938);
#107934=AXIS2_PLACEMENT_3D('',#242499,#133939,#133940);
#107935=AXIS2_PLACEMENT_3D('',#242512,#133941,#133942);
#107936=AXIS2_PLACEMENT_3D('',#242513,#133943,#133944);
#107937=AXIS2_PLACEMENT_3D('',#242514,#133945,#133946);
#107938=AXIS2_PLACEMENT_3D('',#242515,#133947,#133948);
#107939=AXIS2_PLACEMENT_3D('',#242516,#133949,#133950);
#107940=AXIS2_PLACEMENT_3D('',#242535,#133951,#133952);
#107941=AXIS2_PLACEMENT_3D('',#242536,#133953,#133954);
#107942=AXIS2_PLACEMENT_3D('',#242537,#133955,#133956);
#107943=AXIS2_PLACEMENT_3D('',#242538,#133957,#133958);
#107944=AXIS2_PLACEMENT_3D('',#242539,#133959,#133960);
#107945=AXIS2_PLACEMENT_3D('',#242552,#133961,#133962);
#107946=AXIS2_PLACEMENT_3D('',#242565,#133963,#133964);
#107947=AXIS2_PLACEMENT_3D('',#242566,#133965,#133966);
#107948=AXIS2_PLACEMENT_3D('',#242567,#133967,#133968);
#107949=AXIS2_PLACEMENT_3D('',#242568,#133969,#133970);
#107950=AXIS2_PLACEMENT_3D('',#242569,#133971,#133972);
#107951=AXIS2_PLACEMENT_3D('',#242582,#133973,#133974);
#107952=AXIS2_PLACEMENT_3D('',#242583,#133975,#133976);
#107953=AXIS2_PLACEMENT_3D('',#242584,#133977,#133978);
#107954=AXIS2_PLACEMENT_3D('',#242585,#133979,#133980);
#107955=AXIS2_PLACEMENT_3D('',#242586,#133981,#133982);
#107956=AXIS2_PLACEMENT_3D('',#242599,#133983,#133984);
#107957=AXIS2_PLACEMENT_3D('',#242600,#133985,#133986);
#107958=AXIS2_PLACEMENT_3D('',#242601,#133987,#133988);
#107959=AXIS2_PLACEMENT_3D('',#242602,#133989,#133990);
#107960=AXIS2_PLACEMENT_3D('',#242603,#133991,#133992);
#107961=AXIS2_PLACEMENT_3D('',#242616,#133993,#133994);
#107962=AXIS2_PLACEMENT_3D('',#242629,#133995,#133996);
#107963=AXIS2_PLACEMENT_3D('',#242630,#133997,#133998);
#107964=AXIS2_PLACEMENT_3D('',#242631,#133999,#134000);
#107965=AXIS2_PLACEMENT_3D('',#242632,#134001,#134002);
#107966=AXIS2_PLACEMENT_3D('',#242633,#134003,#134004);
#107967=AXIS2_PLACEMENT_3D('',#242652,#134005,#134006);
#107968=AXIS2_PLACEMENT_3D('',#242653,#134007,#134008);
#107969=AXIS2_PLACEMENT_3D('',#242654,#134009,#134010);
#107970=AXIS2_PLACEMENT_3D('',#242655,#134011,#134012);
#107971=AXIS2_PLACEMENT_3D('',#242656,#134013,#134014);
#107972=AXIS2_PLACEMENT_3D('',#242669,#134015,#134016);
#107973=AXIS2_PLACEMENT_3D('',#242688,#134017,#134018);
#107974=AXIS2_PLACEMENT_3D('',#242689,#134019,#134020);
#107975=AXIS2_PLACEMENT_3D('',#242690,#134021,#134022);
#107976=AXIS2_PLACEMENT_3D('',#242691,#134023,#134024);
#107977=AXIS2_PLACEMENT_3D('',#242692,#134025,#134026);
#107978=AXIS2_PLACEMENT_3D('',#242711,#134027,#134028);
#107979=AXIS2_PLACEMENT_3D('',#242724,#134029,#134030);
#107980=AXIS2_PLACEMENT_3D('',#242725,#134031,#134032);
#107981=AXIS2_PLACEMENT_3D('',#242726,#134033,#134034);
#107982=AXIS2_PLACEMENT_3D('',#242727,#134035,#134036);
#107983=AXIS2_PLACEMENT_3D('',#242728,#134037,#134038);
#107984=AXIS2_PLACEMENT_3D('',#242747,#134039,#134040);
#107985=AXIS2_PLACEMENT_3D('',#242748,#134041,#134042);
#107986=AXIS2_PLACEMENT_3D('',#242749,#134043,#134044);
#107987=AXIS2_PLACEMENT_3D('',#242750,#134045,#134046);
#107988=AXIS2_PLACEMENT_3D('',#242751,#134047,#134048);
#107989=AXIS2_PLACEMENT_3D('',#242764,#134049,#134050);
#107990=AXIS2_PLACEMENT_3D('',#242777,#134051,#134052);
#107991=AXIS2_PLACEMENT_3D('',#242778,#134053,#134054);
#107992=AXIS2_PLACEMENT_3D('',#242779,#134055,#134056);
#107993=AXIS2_PLACEMENT_3D('',#242780,#134057,#134058);
#107994=AXIS2_PLACEMENT_3D('',#242781,#134059,#134060);
#107995=AXIS2_PLACEMENT_3D('',#242794,#134061,#134062);
#107996=AXIS2_PLACEMENT_3D('',#242795,#134063,#134064);
#107997=AXIS2_PLACEMENT_3D('',#242796,#134065,#134066);
#107998=AXIS2_PLACEMENT_3D('',#242797,#134067,#134068);
#107999=AXIS2_PLACEMENT_3D('',#242798,#134069,#134070);
#108000=AXIS2_PLACEMENT_3D('',#242811,#134071,#134072);
#108001=AXIS2_PLACEMENT_3D('',#242812,#134073,#134074);
#108002=AXIS2_PLACEMENT_3D('',#242813,#134075,#134076);
#108003=AXIS2_PLACEMENT_3D('',#242814,#134077,#134078);
#108004=AXIS2_PLACEMENT_3D('',#242815,#134079,#134080);
#108005=AXIS2_PLACEMENT_3D('',#242828,#134081,#134082);
#108006=AXIS2_PLACEMENT_3D('',#242841,#134083,#134084);
#108007=AXIS2_PLACEMENT_3D('',#242842,#134085,#134086);
#108008=AXIS2_PLACEMENT_3D('',#242843,#134087,#134088);
#108009=AXIS2_PLACEMENT_3D('',#242844,#134089,#134090);
#108010=AXIS2_PLACEMENT_3D('',#242845,#134091,#134092);
#108011=AXIS2_PLACEMENT_3D('',#242864,#134093,#134094);
#108012=AXIS2_PLACEMENT_3D('',#242865,#134095,#134096);
#108013=AXIS2_PLACEMENT_3D('',#242866,#134097,#134098);
#108014=AXIS2_PLACEMENT_3D('',#242867,#134099,#134100);
#108015=AXIS2_PLACEMENT_3D('',#242868,#134101,#134102);
#108016=AXIS2_PLACEMENT_3D('',#242881,#134103,#134104);
#108017=AXIS2_PLACEMENT_3D('',#242900,#134105,#134106);
#108018=AXIS2_PLACEMENT_3D('',#242901,#134107,#134108);
#108019=AXIS2_PLACEMENT_3D('',#242902,#134109,#134110);
#108020=AXIS2_PLACEMENT_3D('',#242903,#134111,#134112);
#108021=AXIS2_PLACEMENT_3D('',#242904,#134113,#134114);
#108022=AXIS2_PLACEMENT_3D('',#242923,#134115,#134116);
#108023=AXIS2_PLACEMENT_3D('',#242936,#134117,#134118);
#108024=AXIS2_PLACEMENT_3D('',#242937,#134119,#134120);
#108025=AXIS2_PLACEMENT_3D('',#242938,#134121,#134122);
#108026=AXIS2_PLACEMENT_3D('',#242939,#134123,#134124);
#108027=AXIS2_PLACEMENT_3D('',#242940,#134125,#134126);
#108028=AXIS2_PLACEMENT_3D('',#242959,#134127,#134128);
#108029=AXIS2_PLACEMENT_3D('',#242960,#134129,#134130);
#108030=AXIS2_PLACEMENT_3D('',#242961,#134131,#134132);
#108031=AXIS2_PLACEMENT_3D('',#242962,#134133,#134134);
#108032=AXIS2_PLACEMENT_3D('',#242963,#134135,#134136);
#108033=AXIS2_PLACEMENT_3D('',#242976,#134137,#134138);
#108034=AXIS2_PLACEMENT_3D('',#242989,#134139,#134140);
#108035=AXIS2_PLACEMENT_3D('',#242990,#134141,#134142);
#108036=AXIS2_PLACEMENT_3D('',#242991,#134143,#134144);
#108037=AXIS2_PLACEMENT_3D('',#242992,#134145,#134146);
#108038=AXIS2_PLACEMENT_3D('',#242993,#134147,#134148);
#108039=AXIS2_PLACEMENT_3D('',#243006,#134149,#134150);
#108040=AXIS2_PLACEMENT_3D('',#243007,#134151,#134152);
#108041=AXIS2_PLACEMENT_3D('',#243008,#134153,#134154);
#108042=AXIS2_PLACEMENT_3D('',#243009,#134155,#134156);
#108043=AXIS2_PLACEMENT_3D('',#243010,#134157,#134158);
#108044=AXIS2_PLACEMENT_3D('',#243023,#134159,#134160);
#108045=AXIS2_PLACEMENT_3D('',#243024,#134161,#134162);
#108046=AXIS2_PLACEMENT_3D('',#243025,#134163,#134164);
#108047=AXIS2_PLACEMENT_3D('',#243026,#134165,#134166);
#108048=AXIS2_PLACEMENT_3D('',#243027,#134167,#134168);
#108049=AXIS2_PLACEMENT_3D('',#243040,#134169,#134170);
#108050=AXIS2_PLACEMENT_3D('',#243053,#134171,#134172);
#108051=AXIS2_PLACEMENT_3D('',#243054,#134173,#134174);
#108052=AXIS2_PLACEMENT_3D('',#243055,#134175,#134176);
#108053=AXIS2_PLACEMENT_3D('',#243056,#134177,#134178);
#108054=AXIS2_PLACEMENT_3D('',#243057,#134179,#134180);
#108055=AXIS2_PLACEMENT_3D('',#243076,#134181,#134182);
#108056=AXIS2_PLACEMENT_3D('',#243077,#134183,#134184);
#108057=AXIS2_PLACEMENT_3D('',#243078,#134185,#134186);
#108058=AXIS2_PLACEMENT_3D('',#243079,#134187,#134188);
#108059=AXIS2_PLACEMENT_3D('',#243080,#134189,#134190);
#108060=AXIS2_PLACEMENT_3D('',#243093,#134191,#134192);
#108061=AXIS2_PLACEMENT_3D('',#243112,#134193,#134194);
#108062=AXIS2_PLACEMENT_3D('',#243113,#134195,#134196);
#108063=AXIS2_PLACEMENT_3D('',#243114,#134197,#134198);
#108064=AXIS2_PLACEMENT_3D('',#243115,#134199,#134200);
#108065=AXIS2_PLACEMENT_3D('',#243116,#134201,#134202);
#108066=AXIS2_PLACEMENT_3D('',#243135,#134203,#134204);
#108067=AXIS2_PLACEMENT_3D('',#243148,#134205,#134206);
#108068=AXIS2_PLACEMENT_3D('',#243149,#134207,#134208);
#108069=AXIS2_PLACEMENT_3D('',#243150,#134209,#134210);
#108070=AXIS2_PLACEMENT_3D('',#243151,#134211,#134212);
#108071=AXIS2_PLACEMENT_3D('',#243152,#134213,#134214);
#108072=AXIS2_PLACEMENT_3D('',#243171,#134215,#134216);
#108073=AXIS2_PLACEMENT_3D('',#243172,#134217,#134218);
#108074=AXIS2_PLACEMENT_3D('',#243173,#134219,#134220);
#108075=AXIS2_PLACEMENT_3D('',#243174,#134221,#134222);
#108076=AXIS2_PLACEMENT_3D('',#243175,#134223,#134224);
#108077=AXIS2_PLACEMENT_3D('',#243188,#134225,#134226);
#108078=AXIS2_PLACEMENT_3D('',#243201,#134227,#134228);
#108079=AXIS2_PLACEMENT_3D('',#243202,#134229,#134230);
#108080=AXIS2_PLACEMENT_3D('',#243203,#134231,#134232);
#108081=AXIS2_PLACEMENT_3D('',#243204,#134233,#134234);
#108082=AXIS2_PLACEMENT_3D('',#243205,#134235,#134236);
#108083=AXIS2_PLACEMENT_3D('',#243218,#134237,#134238);
#108084=AXIS2_PLACEMENT_3D('',#243219,#134239,#134240);
#108085=AXIS2_PLACEMENT_3D('',#243220,#134241,#134242);
#108086=AXIS2_PLACEMENT_3D('',#243221,#134243,#134244);
#108087=AXIS2_PLACEMENT_3D('',#243222,#134245,#134246);
#108088=AXIS2_PLACEMENT_3D('',#243235,#134247,#134248);
#108089=AXIS2_PLACEMENT_3D('',#243236,#134249,#134250);
#108090=AXIS2_PLACEMENT_3D('',#243237,#134251,#134252);
#108091=AXIS2_PLACEMENT_3D('',#243238,#134253,#134254);
#108092=AXIS2_PLACEMENT_3D('',#243239,#134255,#134256);
#108093=AXIS2_PLACEMENT_3D('',#243252,#134257,#134258);
#108094=AXIS2_PLACEMENT_3D('',#243265,#134259,#134260);
#108095=AXIS2_PLACEMENT_3D('',#243266,#134261,#134262);
#108096=AXIS2_PLACEMENT_3D('',#243267,#134263,#134264);
#108097=AXIS2_PLACEMENT_3D('',#243268,#134265,#134266);
#108098=AXIS2_PLACEMENT_3D('',#243269,#134267,#134268);
#108099=AXIS2_PLACEMENT_3D('',#243288,#134269,#134270);
#108100=AXIS2_PLACEMENT_3D('',#243289,#134271,#134272);
#108101=AXIS2_PLACEMENT_3D('',#243290,#134273,#134274);
#108102=AXIS2_PLACEMENT_3D('',#243291,#134275,#134276);
#108103=AXIS2_PLACEMENT_3D('',#243292,#134277,#134278);
#108104=AXIS2_PLACEMENT_3D('',#243305,#134279,#134280);
#108105=AXIS2_PLACEMENT_3D('',#243324,#134281,#134282);
#108106=AXIS2_PLACEMENT_3D('',#243325,#134283,#134284);
#108107=AXIS2_PLACEMENT_3D('',#243326,#134285,#134286);
#108108=AXIS2_PLACEMENT_3D('',#243327,#134287,#134288);
#108109=AXIS2_PLACEMENT_3D('',#243328,#134289,#134290);
#108110=AXIS2_PLACEMENT_3D('',#243347,#134291,#134292);
#108111=AXIS2_PLACEMENT_3D('',#243360,#134293,#134294);
#108112=AXIS2_PLACEMENT_3D('',#243361,#134295,#134296);
#108113=AXIS2_PLACEMENT_3D('',#243362,#134297,#134298);
#108114=AXIS2_PLACEMENT_3D('',#243363,#134299,#134300);
#108115=AXIS2_PLACEMENT_3D('',#243364,#134301,#134302);
#108116=AXIS2_PLACEMENT_3D('',#243383,#134303,#134304);
#108117=AXIS2_PLACEMENT_3D('',#243384,#134305,#134306);
#108118=AXIS2_PLACEMENT_3D('',#243385,#134307,#134308);
#108119=AXIS2_PLACEMENT_3D('',#243386,#134309,#134310);
#108120=AXIS2_PLACEMENT_3D('',#243387,#134311,#134312);
#108121=AXIS2_PLACEMENT_3D('',#243400,#134313,#134314);
#108122=AXIS2_PLACEMENT_3D('',#243413,#134315,#134316);
#108123=AXIS2_PLACEMENT_3D('',#243414,#134317,#134318);
#108124=AXIS2_PLACEMENT_3D('',#243415,#134319,#134320);
#108125=AXIS2_PLACEMENT_3D('',#243416,#134321,#134322);
#108126=AXIS2_PLACEMENT_3D('',#243417,#134323,#134324);
#108127=AXIS2_PLACEMENT_3D('',#243430,#134325,#134326);
#108128=AXIS2_PLACEMENT_3D('',#243431,#134327,#134328);
#108129=AXIS2_PLACEMENT_3D('',#243432,#134329,#134330);
#108130=AXIS2_PLACEMENT_3D('',#243433,#134331,#134332);
#108131=AXIS2_PLACEMENT_3D('',#243434,#134333,#134334);
#108132=AXIS2_PLACEMENT_3D('',#243447,#134335,#134336);
#108133=AXIS2_PLACEMENT_3D('',#243448,#134337,#134338);
#108134=AXIS2_PLACEMENT_3D('',#243449,#134339,#134340);
#108135=AXIS2_PLACEMENT_3D('',#243450,#134341,#134342);
#108136=AXIS2_PLACEMENT_3D('',#243451,#134343,#134344);
#108137=AXIS2_PLACEMENT_3D('',#243464,#134345,#134346);
#108138=AXIS2_PLACEMENT_3D('',#243477,#134347,#134348);
#108139=AXIS2_PLACEMENT_3D('',#243478,#134349,#134350);
#108140=AXIS2_PLACEMENT_3D('',#243479,#134351,#134352);
#108141=AXIS2_PLACEMENT_3D('',#243480,#134353,#134354);
#108142=AXIS2_PLACEMENT_3D('',#243481,#134355,#134356);
#108143=AXIS2_PLACEMENT_3D('',#243500,#134357,#134358);
#108144=AXIS2_PLACEMENT_3D('',#243501,#134359,#134360);
#108145=AXIS2_PLACEMENT_3D('',#243502,#134361,#134362);
#108146=AXIS2_PLACEMENT_3D('',#243503,#134363,#134364);
#108147=AXIS2_PLACEMENT_3D('',#243504,#134365,#134366);
#108148=AXIS2_PLACEMENT_3D('',#243517,#134367,#134368);
#108149=AXIS2_PLACEMENT_3D('',#243536,#134369,#134370);
#108150=AXIS2_PLACEMENT_3D('',#243537,#134371,#134372);
#108151=AXIS2_PLACEMENT_3D('',#243538,#134373,#134374);
#108152=AXIS2_PLACEMENT_3D('',#243539,#134375,#134376);
#108153=AXIS2_PLACEMENT_3D('',#243540,#134377,#134378);
#108154=AXIS2_PLACEMENT_3D('',#243559,#134379,#134380);
#108155=AXIS2_PLACEMENT_3D('',#243572,#134381,#134382);
#108156=AXIS2_PLACEMENT_3D('',#243573,#134383,#134384);
#108157=AXIS2_PLACEMENT_3D('',#243574,#134385,#134386);
#108158=AXIS2_PLACEMENT_3D('',#243575,#134387,#134388);
#108159=AXIS2_PLACEMENT_3D('',#243576,#134389,#134390);
#108160=AXIS2_PLACEMENT_3D('',#243595,#134391,#134392);
#108161=AXIS2_PLACEMENT_3D('',#243596,#134393,#134394);
#108162=AXIS2_PLACEMENT_3D('',#243597,#134395,#134396);
#108163=AXIS2_PLACEMENT_3D('',#243598,#134397,#134398);
#108164=AXIS2_PLACEMENT_3D('',#243599,#134399,#134400);
#108165=AXIS2_PLACEMENT_3D('',#243612,#134401,#134402);
#108166=AXIS2_PLACEMENT_3D('',#243625,#134403,#134404);
#108167=AXIS2_PLACEMENT_3D('',#243626,#134405,#134406);
#108168=AXIS2_PLACEMENT_3D('',#243627,#134407,#134408);
#108169=AXIS2_PLACEMENT_3D('',#243628,#134409,#134410);
#108170=AXIS2_PLACEMENT_3D('',#243629,#134411,#134412);
#108171=AXIS2_PLACEMENT_3D('',#243642,#134413,#134414);
#108172=AXIS2_PLACEMENT_3D('',#243643,#134415,#134416);
#108173=AXIS2_PLACEMENT_3D('',#243644,#134417,#134418);
#108174=AXIS2_PLACEMENT_3D('',#243645,#134419,#134420);
#108175=AXIS2_PLACEMENT_3D('',#243646,#134421,#134422);
#108176=AXIS2_PLACEMENT_3D('',#243659,#134423,#134424);
#108177=AXIS2_PLACEMENT_3D('',#243660,#134425,#134426);
#108178=AXIS2_PLACEMENT_3D('',#243661,#134427,#134428);
#108179=AXIS2_PLACEMENT_3D('',#243662,#134429,#134430);
#108180=AXIS2_PLACEMENT_3D('',#243663,#134431,#134432);
#108181=AXIS2_PLACEMENT_3D('',#243676,#134433,#134434);
#108182=AXIS2_PLACEMENT_3D('',#243689,#134435,#134436);
#108183=AXIS2_PLACEMENT_3D('',#243690,#134437,#134438);
#108184=AXIS2_PLACEMENT_3D('',#243691,#134439,#134440);
#108185=AXIS2_PLACEMENT_3D('',#243692,#134441,#134442);
#108186=AXIS2_PLACEMENT_3D('',#243693,#134443,#134444);
#108187=AXIS2_PLACEMENT_3D('',#243712,#134445,#134446);
#108188=AXIS2_PLACEMENT_3D('',#243713,#134447,#134448);
#108189=AXIS2_PLACEMENT_3D('',#243714,#134449,#134450);
#108190=AXIS2_PLACEMENT_3D('',#243715,#134451,#134452);
#108191=AXIS2_PLACEMENT_3D('',#243716,#134453,#134454);
#108192=AXIS2_PLACEMENT_3D('',#243729,#134455,#134456);
#108193=AXIS2_PLACEMENT_3D('',#243748,#134457,#134458);
#108194=AXIS2_PLACEMENT_3D('',#243749,#134459,#134460);
#108195=AXIS2_PLACEMENT_3D('',#243750,#134461,#134462);
#108196=AXIS2_PLACEMENT_3D('',#243751,#134463,#134464);
#108197=AXIS2_PLACEMENT_3D('',#243752,#134465,#134466);
#108198=AXIS2_PLACEMENT_3D('',#243771,#134467,#134468);
#108199=AXIS2_PLACEMENT_3D('',#243784,#134469,#134470);
#108200=AXIS2_PLACEMENT_3D('',#243785,#134471,#134472);
#108201=AXIS2_PLACEMENT_3D('',#243786,#134473,#134474);
#108202=AXIS2_PLACEMENT_3D('',#243787,#134475,#134476);
#108203=AXIS2_PLACEMENT_3D('',#243788,#134477,#134478);
#108204=AXIS2_PLACEMENT_3D('',#243807,#134479,#134480);
#108205=AXIS2_PLACEMENT_3D('',#243808,#134481,#134482);
#108206=AXIS2_PLACEMENT_3D('',#243809,#134483,#134484);
#108207=AXIS2_PLACEMENT_3D('',#243810,#134485,#134486);
#108208=AXIS2_PLACEMENT_3D('',#243811,#134487,#134488);
#108209=AXIS2_PLACEMENT_3D('',#243824,#134489,#134490);
#108210=AXIS2_PLACEMENT_3D('',#243837,#134491,#134492);
#108211=AXIS2_PLACEMENT_3D('',#243838,#134493,#134494);
#108212=AXIS2_PLACEMENT_3D('',#243839,#134495,#134496);
#108213=AXIS2_PLACEMENT_3D('',#243840,#134497,#134498);
#108214=AXIS2_PLACEMENT_3D('',#243841,#134499,#134500);
#108215=AXIS2_PLACEMENT_3D('',#243854,#134501,#134502);
#108216=AXIS2_PLACEMENT_3D('',#243855,#134503,#134504);
#108217=AXIS2_PLACEMENT_3D('',#243856,#134505,#134506);
#108218=AXIS2_PLACEMENT_3D('',#243857,#134507,#134508);
#108219=AXIS2_PLACEMENT_3D('',#243858,#134509,#134510);
#108220=AXIS2_PLACEMENT_3D('',#243871,#134511,#134512);
#108221=AXIS2_PLACEMENT_3D('',#243872,#134513,#134514);
#108222=AXIS2_PLACEMENT_3D('',#243873,#134515,#134516);
#108223=AXIS2_PLACEMENT_3D('',#243874,#134517,#134518);
#108224=AXIS2_PLACEMENT_3D('',#243875,#134519,#134520);
#108225=AXIS2_PLACEMENT_3D('',#243888,#134521,#134522);
#108226=AXIS2_PLACEMENT_3D('',#243901,#134523,#134524);
#108227=AXIS2_PLACEMENT_3D('',#243902,#134525,#134526);
#108228=AXIS2_PLACEMENT_3D('',#243903,#134527,#134528);
#108229=AXIS2_PLACEMENT_3D('',#243904,#134529,#134530);
#108230=AXIS2_PLACEMENT_3D('',#243905,#134531,#134532);
#108231=AXIS2_PLACEMENT_3D('',#243924,#134533,#134534);
#108232=AXIS2_PLACEMENT_3D('',#243925,#134535,#134536);
#108233=AXIS2_PLACEMENT_3D('',#243926,#134537,#134538);
#108234=AXIS2_PLACEMENT_3D('',#243927,#134539,#134540);
#108235=AXIS2_PLACEMENT_3D('',#243928,#134541,#134542);
#108236=AXIS2_PLACEMENT_3D('',#243941,#134543,#134544);
#108237=AXIS2_PLACEMENT_3D('',#243960,#134545,#134546);
#108238=AXIS2_PLACEMENT_3D('',#243961,#134547,#134548);
#108239=AXIS2_PLACEMENT_3D('',#243962,#134549,#134550);
#108240=AXIS2_PLACEMENT_3D('',#243963,#134551,#134552);
#108241=AXIS2_PLACEMENT_3D('',#243964,#134553,#134554);
#108242=AXIS2_PLACEMENT_3D('',#243983,#134555,#134556);
#108243=AXIS2_PLACEMENT_3D('',#243996,#134557,#134558);
#108244=AXIS2_PLACEMENT_3D('',#243997,#134559,#134560);
#108245=AXIS2_PLACEMENT_3D('',#243998,#134561,#134562);
#108246=AXIS2_PLACEMENT_3D('',#243999,#134563,#134564);
#108247=AXIS2_PLACEMENT_3D('',#244000,#134565,#134566);
#108248=AXIS2_PLACEMENT_3D('',#244019,#134567,#134568);
#108249=AXIS2_PLACEMENT_3D('',#244020,#134569,#134570);
#108250=AXIS2_PLACEMENT_3D('',#244021,#134571,#134572);
#108251=AXIS2_PLACEMENT_3D('',#244022,#134573,#134574);
#108252=AXIS2_PLACEMENT_3D('',#244023,#134575,#134576);
#108253=AXIS2_PLACEMENT_3D('',#244036,#134577,#134578);
#108254=AXIS2_PLACEMENT_3D('',#244049,#134579,#134580);
#108255=AXIS2_PLACEMENT_3D('',#244050,#134581,#134582);
#108256=AXIS2_PLACEMENT_3D('',#244051,#134583,#134584);
#108257=AXIS2_PLACEMENT_3D('',#244052,#134585,#134586);
#108258=AXIS2_PLACEMENT_3D('',#244053,#134587,#134588);
#108259=AXIS2_PLACEMENT_3D('',#244066,#134589,#134590);
#108260=AXIS2_PLACEMENT_3D('',#244067,#134591,#134592);
#108261=AXIS2_PLACEMENT_3D('',#244068,#134593,#134594);
#108262=AXIS2_PLACEMENT_3D('',#244069,#134595,#134596);
#108263=AXIS2_PLACEMENT_3D('',#244070,#134597,#134598);
#108264=AXIS2_PLACEMENT_3D('',#244083,#134599,#134600);
#108265=AXIS2_PLACEMENT_3D('',#244084,#134601,#134602);
#108266=AXIS2_PLACEMENT_3D('',#244085,#134603,#134604);
#108267=AXIS2_PLACEMENT_3D('',#244086,#134605,#134606);
#108268=AXIS2_PLACEMENT_3D('',#244087,#134607,#134608);
#108269=AXIS2_PLACEMENT_3D('',#244100,#134609,#134610);
#108270=AXIS2_PLACEMENT_3D('',#244113,#134611,#134612);
#108271=AXIS2_PLACEMENT_3D('',#244114,#134613,#134614);
#108272=AXIS2_PLACEMENT_3D('',#244115,#134615,#134616);
#108273=AXIS2_PLACEMENT_3D('',#244116,#134617,#134618);
#108274=AXIS2_PLACEMENT_3D('',#244117,#134619,#134620);
#108275=AXIS2_PLACEMENT_3D('',#244136,#134621,#134622);
#108276=AXIS2_PLACEMENT_3D('',#244137,#134623,#134624);
#108277=AXIS2_PLACEMENT_3D('',#244138,#134625,#134626);
#108278=AXIS2_PLACEMENT_3D('',#244139,#134627,#134628);
#108279=AXIS2_PLACEMENT_3D('',#244140,#134629,#134630);
#108280=AXIS2_PLACEMENT_3D('',#244153,#134631,#134632);
#108281=AXIS2_PLACEMENT_3D('',#244172,#134633,#134634);
#108282=AXIS2_PLACEMENT_3D('',#244173,#134635,#134636);
#108283=AXIS2_PLACEMENT_3D('',#244174,#134637,#134638);
#108284=AXIS2_PLACEMENT_3D('',#244175,#134639,#134640);
#108285=AXIS2_PLACEMENT_3D('',#244176,#134641,#134642);
#108286=AXIS2_PLACEMENT_3D('',#244195,#134643,#134644);
#108287=AXIS2_PLACEMENT_3D('',#244208,#134645,#134646);
#108288=AXIS2_PLACEMENT_3D('',#244209,#134647,#134648);
#108289=AXIS2_PLACEMENT_3D('',#244210,#134649,#134650);
#108290=AXIS2_PLACEMENT_3D('',#244211,#134651,#134652);
#108291=AXIS2_PLACEMENT_3D('',#244212,#134653,#134654);
#108292=AXIS2_PLACEMENT_3D('',#244231,#134655,#134656);
#108293=AXIS2_PLACEMENT_3D('',#244232,#134657,#134658);
#108294=AXIS2_PLACEMENT_3D('',#244233,#134659,#134660);
#108295=AXIS2_PLACEMENT_3D('',#244234,#134661,#134662);
#108296=AXIS2_PLACEMENT_3D('',#244235,#134663,#134664);
#108297=AXIS2_PLACEMENT_3D('',#244248,#134665,#134666);
#108298=AXIS2_PLACEMENT_3D('',#244261,#134667,#134668);
#108299=AXIS2_PLACEMENT_3D('',#244262,#134669,#134670);
#108300=AXIS2_PLACEMENT_3D('',#244263,#134671,#134672);
#108301=AXIS2_PLACEMENT_3D('',#244264,#134673,#134674);
#108302=AXIS2_PLACEMENT_3D('',#244265,#134675,#134676);
#108303=AXIS2_PLACEMENT_3D('',#244278,#134677,#134678);
#108304=AXIS2_PLACEMENT_3D('',#244279,#134679,#134680);
#108305=AXIS2_PLACEMENT_3D('',#244280,#134681,#134682);
#108306=AXIS2_PLACEMENT_3D('',#244281,#134683,#134684);
#108307=AXIS2_PLACEMENT_3D('',#244282,#134685,#134686);
#108308=AXIS2_PLACEMENT_3D('',#244295,#134687,#134688);
#108309=AXIS2_PLACEMENT_3D('',#244296,#134689,#134690);
#108310=AXIS2_PLACEMENT_3D('',#244297,#134691,#134692);
#108311=AXIS2_PLACEMENT_3D('',#244298,#134693,#134694);
#108312=AXIS2_PLACEMENT_3D('',#244299,#134695,#134696);
#108313=AXIS2_PLACEMENT_3D('',#244312,#134697,#134698);
#108314=AXIS2_PLACEMENT_3D('',#244325,#134699,#134700);
#108315=AXIS2_PLACEMENT_3D('',#244326,#134701,#134702);
#108316=AXIS2_PLACEMENT_3D('',#244327,#134703,#134704);
#108317=AXIS2_PLACEMENT_3D('',#244328,#134705,#134706);
#108318=AXIS2_PLACEMENT_3D('',#244329,#134707,#134708);
#108319=AXIS2_PLACEMENT_3D('',#244348,#134709,#134710);
#108320=AXIS2_PLACEMENT_3D('',#244349,#134711,#134712);
#108321=AXIS2_PLACEMENT_3D('',#244350,#134713,#134714);
#108322=AXIS2_PLACEMENT_3D('',#244351,#134715,#134716);
#108323=AXIS2_PLACEMENT_3D('',#244352,#134717,#134718);
#108324=AXIS2_PLACEMENT_3D('',#244365,#134719,#134720);
#108325=AXIS2_PLACEMENT_3D('',#244384,#134721,#134722);
#108326=AXIS2_PLACEMENT_3D('',#244385,#134723,#134724);
#108327=AXIS2_PLACEMENT_3D('',#244386,#134725,#134726);
#108328=AXIS2_PLACEMENT_3D('',#244387,#134727,#134728);
#108329=AXIS2_PLACEMENT_3D('',#244388,#134729,#134730);
#108330=AXIS2_PLACEMENT_3D('',#244407,#134731,#134732);
#108331=AXIS2_PLACEMENT_3D('',#244420,#134733,#134734);
#108332=AXIS2_PLACEMENT_3D('',#244421,#134735,#134736);
#108333=AXIS2_PLACEMENT_3D('',#244422,#134737,#134738);
#108334=AXIS2_PLACEMENT_3D('',#244423,#134739,#134740);
#108335=AXIS2_PLACEMENT_3D('',#244424,#134741,#134742);
#108336=AXIS2_PLACEMENT_3D('',#244443,#134743,#134744);
#108337=AXIS2_PLACEMENT_3D('',#244444,#134745,#134746);
#108338=AXIS2_PLACEMENT_3D('',#244445,#134747,#134748);
#108339=AXIS2_PLACEMENT_3D('',#244446,#134749,#134750);
#108340=AXIS2_PLACEMENT_3D('',#244447,#134751,#134752);
#108341=AXIS2_PLACEMENT_3D('',#244460,#134753,#134754);
#108342=AXIS2_PLACEMENT_3D('',#244473,#134755,#134756);
#108343=AXIS2_PLACEMENT_3D('',#244474,#134757,#134758);
#108344=AXIS2_PLACEMENT_3D('',#244475,#134759,#134760);
#108345=AXIS2_PLACEMENT_3D('',#244476,#134761,#134762);
#108346=AXIS2_PLACEMENT_3D('',#244477,#134763,#134764);
#108347=AXIS2_PLACEMENT_3D('',#244490,#134765,#134766);
#108348=AXIS2_PLACEMENT_3D('',#244491,#134767,#134768);
#108349=AXIS2_PLACEMENT_3D('',#244492,#134769,#134770);
#108350=AXIS2_PLACEMENT_3D('',#244493,#134771,#134772);
#108351=AXIS2_PLACEMENT_3D('',#244494,#134773,#134774);
#108352=AXIS2_PLACEMENT_3D('',#244507,#134775,#134776);
#108353=AXIS2_PLACEMENT_3D('',#244508,#134777,#134778);
#108354=AXIS2_PLACEMENT_3D('',#244509,#134779,#134780);
#108355=AXIS2_PLACEMENT_3D('',#244510,#134781,#134782);
#108356=AXIS2_PLACEMENT_3D('',#244511,#134783,#134784);
#108357=AXIS2_PLACEMENT_3D('',#244524,#134785,#134786);
#108358=AXIS2_PLACEMENT_3D('',#244537,#134787,#134788);
#108359=AXIS2_PLACEMENT_3D('',#244538,#134789,#134790);
#108360=AXIS2_PLACEMENT_3D('',#244539,#134791,#134792);
#108361=AXIS2_PLACEMENT_3D('',#244540,#134793,#134794);
#108362=AXIS2_PLACEMENT_3D('',#244541,#134795,#134796);
#108363=AXIS2_PLACEMENT_3D('',#244560,#134797,#134798);
#108364=AXIS2_PLACEMENT_3D('',#244561,#134799,#134800);
#108365=AXIS2_PLACEMENT_3D('',#244562,#134801,#134802);
#108366=AXIS2_PLACEMENT_3D('',#244563,#134803,#134804);
#108367=AXIS2_PLACEMENT_3D('',#244564,#134805,#134806);
#108368=AXIS2_PLACEMENT_3D('',#244577,#134807,#134808);
#108369=AXIS2_PLACEMENT_3D('',#244596,#134809,#134810);
#108370=AXIS2_PLACEMENT_3D('',#244597,#134811,#134812);
#108371=AXIS2_PLACEMENT_3D('',#244598,#134813,#134814);
#108372=AXIS2_PLACEMENT_3D('',#244599,#134815,#134816);
#108373=AXIS2_PLACEMENT_3D('',#244600,#134817,#134818);
#108374=AXIS2_PLACEMENT_3D('',#244619,#134819,#134820);
#108375=AXIS2_PLACEMENT_3D('',#244632,#134821,#134822);
#108376=AXIS2_PLACEMENT_3D('',#244633,#134823,#134824);
#108377=AXIS2_PLACEMENT_3D('',#244634,#134825,#134826);
#108378=AXIS2_PLACEMENT_3D('',#244635,#134827,#134828);
#108379=AXIS2_PLACEMENT_3D('',#244636,#134829,#134830);
#108380=AXIS2_PLACEMENT_3D('',#244655,#134831,#134832);
#108381=AXIS2_PLACEMENT_3D('',#244656,#134833,#134834);
#108382=AXIS2_PLACEMENT_3D('',#244657,#134835,#134836);
#108383=AXIS2_PLACEMENT_3D('',#244658,#134837,#134838);
#108384=AXIS2_PLACEMENT_3D('',#244659,#134839,#134840);
#108385=AXIS2_PLACEMENT_3D('',#244672,#134841,#134842);
#108386=AXIS2_PLACEMENT_3D('',#244685,#134843,#134844);
#108387=AXIS2_PLACEMENT_3D('',#244686,#134845,#134846);
#108388=AXIS2_PLACEMENT_3D('',#244687,#134847,#134848);
#108389=AXIS2_PLACEMENT_3D('',#244688,#134849,#134850);
#108390=AXIS2_PLACEMENT_3D('',#244689,#134851,#134852);
#108391=AXIS2_PLACEMENT_3D('',#244702,#134853,#134854);
#108392=AXIS2_PLACEMENT_3D('',#244703,#134855,#134856);
#108393=AXIS2_PLACEMENT_3D('',#244704,#134857,#134858);
#108394=AXIS2_PLACEMENT_3D('',#244705,#134859,#134860);
#108395=AXIS2_PLACEMENT_3D('',#244706,#134861,#134862);
#108396=AXIS2_PLACEMENT_3D('',#244719,#134863,#134864);
#108397=AXIS2_PLACEMENT_3D('',#244720,#134865,#134866);
#108398=AXIS2_PLACEMENT_3D('',#244721,#134867,#134868);
#108399=AXIS2_PLACEMENT_3D('',#244722,#134869,#134870);
#108400=AXIS2_PLACEMENT_3D('',#244723,#134871,#134872);
#108401=AXIS2_PLACEMENT_3D('',#244736,#134873,#134874);
#108402=AXIS2_PLACEMENT_3D('',#244749,#134875,#134876);
#108403=AXIS2_PLACEMENT_3D('',#244750,#134877,#134878);
#108404=AXIS2_PLACEMENT_3D('',#244751,#134879,#134880);
#108405=AXIS2_PLACEMENT_3D('',#244752,#134881,#134882);
#108406=AXIS2_PLACEMENT_3D('',#244753,#134883,#134884);
#108407=AXIS2_PLACEMENT_3D('',#244772,#134885,#134886);
#108408=AXIS2_PLACEMENT_3D('',#244773,#134887,#134888);
#108409=AXIS2_PLACEMENT_3D('',#244774,#134889,#134890);
#108410=AXIS2_PLACEMENT_3D('',#244775,#134891,#134892);
#108411=AXIS2_PLACEMENT_3D('',#244776,#134893,#134894);
#108412=AXIS2_PLACEMENT_3D('',#244789,#134895,#134896);
#108413=AXIS2_PLACEMENT_3D('',#244808,#134897,#134898);
#108414=AXIS2_PLACEMENT_3D('',#244809,#134899,#134900);
#108415=AXIS2_PLACEMENT_3D('',#244810,#134901,#134902);
#108416=AXIS2_PLACEMENT_3D('',#244811,#134903,#134904);
#108417=AXIS2_PLACEMENT_3D('',#244812,#134905,#134906);
#108418=AXIS2_PLACEMENT_3D('',#244831,#134907,#134908);
#108419=AXIS2_PLACEMENT_3D('',#244844,#134909,#134910);
#108420=AXIS2_PLACEMENT_3D('',#244845,#134911,#134912);
#108421=AXIS2_PLACEMENT_3D('',#244846,#134913,#134914);
#108422=AXIS2_PLACEMENT_3D('',#244847,#134915,#134916);
#108423=AXIS2_PLACEMENT_3D('',#244848,#134917,#134918);
#108424=AXIS2_PLACEMENT_3D('',#244867,#134919,#134920);
#108425=AXIS2_PLACEMENT_3D('',#244868,#134921,#134922);
#108426=AXIS2_PLACEMENT_3D('',#244869,#134923,#134924);
#108427=AXIS2_PLACEMENT_3D('',#244870,#134925,#134926);
#108428=AXIS2_PLACEMENT_3D('',#244871,#134927,#134928);
#108429=AXIS2_PLACEMENT_3D('',#244884,#134929,#134930);
#108430=AXIS2_PLACEMENT_3D('',#244897,#134931,#134932);
#108431=AXIS2_PLACEMENT_3D('',#244898,#134933,#134934);
#108432=AXIS2_PLACEMENT_3D('',#244899,#134935,#134936);
#108433=AXIS2_PLACEMENT_3D('',#244900,#134937,#134938);
#108434=AXIS2_PLACEMENT_3D('',#244901,#134939,#134940);
#108435=AXIS2_PLACEMENT_3D('',#244914,#134941,#134942);
#108436=AXIS2_PLACEMENT_3D('',#244915,#134943,#134944);
#108437=AXIS2_PLACEMENT_3D('',#244916,#134945,#134946);
#108438=AXIS2_PLACEMENT_3D('',#244917,#134947,#134948);
#108439=AXIS2_PLACEMENT_3D('',#244918,#134949,#134950);
#108440=AXIS2_PLACEMENT_3D('',#244931,#134951,#134952);
#108441=AXIS2_PLACEMENT_3D('',#244932,#134953,#134954);
#108442=AXIS2_PLACEMENT_3D('',#244933,#134955,#134956);
#108443=AXIS2_PLACEMENT_3D('',#244934,#134957,#134958);
#108444=AXIS2_PLACEMENT_3D('',#244935,#134959,#134960);
#108445=AXIS2_PLACEMENT_3D('',#244948,#134961,#134962);
#108446=AXIS2_PLACEMENT_3D('',#244961,#134963,#134964);
#108447=AXIS2_PLACEMENT_3D('',#244962,#134965,#134966);
#108448=AXIS2_PLACEMENT_3D('',#244963,#134967,#134968);
#108449=AXIS2_PLACEMENT_3D('',#244964,#134969,#134970);
#108450=AXIS2_PLACEMENT_3D('',#244965,#134971,#134972);
#108451=AXIS2_PLACEMENT_3D('',#244984,#134973,#134974);
#108452=AXIS2_PLACEMENT_3D('',#244985,#134975,#134976);
#108453=AXIS2_PLACEMENT_3D('',#244986,#134977,#134978);
#108454=AXIS2_PLACEMENT_3D('',#244987,#134979,#134980);
#108455=AXIS2_PLACEMENT_3D('',#244988,#134981,#134982);
#108456=AXIS2_PLACEMENT_3D('',#245001,#134983,#134984);
#108457=AXIS2_PLACEMENT_3D('',#245020,#134985,#134986);
#108458=AXIS2_PLACEMENT_3D('',#245021,#134987,#134988);
#108459=AXIS2_PLACEMENT_3D('',#245022,#134989,#134990);
#108460=AXIS2_PLACEMENT_3D('',#245023,#134991,#134992);
#108461=AXIS2_PLACEMENT_3D('',#245024,#134993,#134994);
#108462=AXIS2_PLACEMENT_3D('',#245043,#134995,#134996);
#108463=AXIS2_PLACEMENT_3D('',#245056,#134997,#134998);
#108464=AXIS2_PLACEMENT_3D('',#245057,#134999,#135000);
#108465=AXIS2_PLACEMENT_3D('',#245058,#135001,#135002);
#108466=AXIS2_PLACEMENT_3D('',#245059,#135003,#135004);
#108467=AXIS2_PLACEMENT_3D('',#245060,#135005,#135006);
#108468=AXIS2_PLACEMENT_3D('',#245079,#135007,#135008);
#108469=AXIS2_PLACEMENT_3D('',#245080,#135009,#135010);
#108470=AXIS2_PLACEMENT_3D('',#245081,#135011,#135012);
#108471=AXIS2_PLACEMENT_3D('',#245082,#135013,#135014);
#108472=AXIS2_PLACEMENT_3D('',#245083,#135015,#135016);
#108473=AXIS2_PLACEMENT_3D('',#245096,#135017,#135018);
#108474=AXIS2_PLACEMENT_3D('',#245109,#135019,#135020);
#108475=AXIS2_PLACEMENT_3D('',#245110,#135021,#135022);
#108476=AXIS2_PLACEMENT_3D('',#245111,#135023,#135024);
#108477=AXIS2_PLACEMENT_3D('',#245112,#135025,#135026);
#108478=AXIS2_PLACEMENT_3D('',#245113,#135027,#135028);
#108479=AXIS2_PLACEMENT_3D('',#245126,#135029,#135030);
#108480=AXIS2_PLACEMENT_3D('',#245127,#135031,#135032);
#108481=AXIS2_PLACEMENT_3D('',#245128,#135033,#135034);
#108482=AXIS2_PLACEMENT_3D('',#245129,#135035,#135036);
#108483=AXIS2_PLACEMENT_3D('',#245130,#135037,#135038);
#108484=AXIS2_PLACEMENT_3D('',#245143,#135039,#135040);
#108485=AXIS2_PLACEMENT_3D('',#245144,#135041,#135042);
#108486=AXIS2_PLACEMENT_3D('',#245145,#135043,#135044);
#108487=AXIS2_PLACEMENT_3D('',#245146,#135045,#135046);
#108488=AXIS2_PLACEMENT_3D('',#245147,#135047,#135048);
#108489=AXIS2_PLACEMENT_3D('',#245160,#135049,#135050);
#108490=AXIS2_PLACEMENT_3D('',#245173,#135051,#135052);
#108491=AXIS2_PLACEMENT_3D('',#245174,#135053,#135054);
#108492=AXIS2_PLACEMENT_3D('',#245175,#135055,#135056);
#108493=AXIS2_PLACEMENT_3D('',#245176,#135057,#135058);
#108494=AXIS2_PLACEMENT_3D('',#245177,#135059,#135060);
#108495=AXIS2_PLACEMENT_3D('',#245196,#135061,#135062);
#108496=AXIS2_PLACEMENT_3D('',#245197,#135063,#135064);
#108497=AXIS2_PLACEMENT_3D('',#245198,#135065,#135066);
#108498=AXIS2_PLACEMENT_3D('',#245199,#135067,#135068);
#108499=AXIS2_PLACEMENT_3D('',#245200,#135069,#135070);
#108500=AXIS2_PLACEMENT_3D('',#245213,#135071,#135072);
#108501=AXIS2_PLACEMENT_3D('',#245232,#135073,#135074);
#108502=AXIS2_PLACEMENT_3D('',#245233,#135075,#135076);
#108503=AXIS2_PLACEMENT_3D('',#245234,#135077,#135078);
#108504=AXIS2_PLACEMENT_3D('',#245235,#135079,#135080);
#108505=AXIS2_PLACEMENT_3D('',#245236,#135081,#135082);
#108506=AXIS2_PLACEMENT_3D('',#245255,#135083,#135084);
#108507=AXIS2_PLACEMENT_3D('',#245268,#135085,#135086);
#108508=AXIS2_PLACEMENT_3D('',#245269,#135087,#135088);
#108509=AXIS2_PLACEMENT_3D('',#245270,#135089,#135090);
#108510=AXIS2_PLACEMENT_3D('',#245271,#135091,#135092);
#108511=AXIS2_PLACEMENT_3D('',#245272,#135093,#135094);
#108512=AXIS2_PLACEMENT_3D('',#245291,#135095,#135096);
#108513=AXIS2_PLACEMENT_3D('',#245292,#135097,#135098);
#108514=AXIS2_PLACEMENT_3D('',#245293,#135099,#135100);
#108515=AXIS2_PLACEMENT_3D('',#245294,#135101,#135102);
#108516=AXIS2_PLACEMENT_3D('',#245295,#135103,#135104);
#108517=AXIS2_PLACEMENT_3D('',#245308,#135105,#135106);
#108518=AXIS2_PLACEMENT_3D('',#245321,#135107,#135108);
#108519=AXIS2_PLACEMENT_3D('',#245322,#135109,#135110);
#108520=AXIS2_PLACEMENT_3D('',#245323,#135111,#135112);
#108521=AXIS2_PLACEMENT_3D('',#245324,#135113,#135114);
#108522=AXIS2_PLACEMENT_3D('',#245325,#135115,#135116);
#108523=AXIS2_PLACEMENT_3D('',#245338,#135117,#135118);
#108524=AXIS2_PLACEMENT_3D('',#245339,#135119,#135120);
#108525=AXIS2_PLACEMENT_3D('',#245340,#135121,#135122);
#108526=AXIS2_PLACEMENT_3D('',#245341,#135123,#135124);
#108527=AXIS2_PLACEMENT_3D('',#245342,#135125,#135126);
#108528=AXIS2_PLACEMENT_3D('',#245355,#135127,#135128);
#108529=AXIS2_PLACEMENT_3D('',#245356,#135129,#135130);
#108530=AXIS2_PLACEMENT_3D('',#245357,#135131,#135132);
#108531=AXIS2_PLACEMENT_3D('',#245358,#135133,#135134);
#108532=AXIS2_PLACEMENT_3D('',#245359,#135135,#135136);
#108533=AXIS2_PLACEMENT_3D('',#245372,#135137,#135138);
#108534=AXIS2_PLACEMENT_3D('',#245385,#135139,#135140);
#108535=AXIS2_PLACEMENT_3D('',#245386,#135141,#135142);
#108536=AXIS2_PLACEMENT_3D('',#245387,#135143,#135144);
#108537=AXIS2_PLACEMENT_3D('',#245388,#135145,#135146);
#108538=AXIS2_PLACEMENT_3D('',#245389,#135147,#135148);
#108539=AXIS2_PLACEMENT_3D('',#245408,#135149,#135150);
#108540=AXIS2_PLACEMENT_3D('',#245409,#135151,#135152);
#108541=AXIS2_PLACEMENT_3D('',#245410,#135153,#135154);
#108542=AXIS2_PLACEMENT_3D('',#245411,#135155,#135156);
#108543=AXIS2_PLACEMENT_3D('',#245412,#135157,#135158);
#108544=AXIS2_PLACEMENT_3D('',#245425,#135159,#135160);
#108545=AXIS2_PLACEMENT_3D('',#245444,#135161,#135162);
#108546=AXIS2_PLACEMENT_3D('',#245445,#135163,#135164);
#108547=AXIS2_PLACEMENT_3D('',#245446,#135165,#135166);
#108548=AXIS2_PLACEMENT_3D('',#245447,#135167,#135168);
#108549=AXIS2_PLACEMENT_3D('',#245448,#135169,#135170);
#108550=AXIS2_PLACEMENT_3D('',#245467,#135171,#135172);
#108551=AXIS2_PLACEMENT_3D('',#245480,#135173,#135174);
#108552=AXIS2_PLACEMENT_3D('',#245481,#135175,#135176);
#108553=AXIS2_PLACEMENT_3D('',#245482,#135177,#135178);
#108554=AXIS2_PLACEMENT_3D('',#245483,#135179,#135180);
#108555=AXIS2_PLACEMENT_3D('',#245484,#135181,#135182);
#108556=AXIS2_PLACEMENT_3D('',#245503,#135183,#135184);
#108557=AXIS2_PLACEMENT_3D('',#245504,#135185,#135186);
#108558=AXIS2_PLACEMENT_3D('',#245505,#135187,#135188);
#108559=AXIS2_PLACEMENT_3D('',#245506,#135189,#135190);
#108560=AXIS2_PLACEMENT_3D('',#245507,#135191,#135192);
#108561=AXIS2_PLACEMENT_3D('',#245520,#135193,#135194);
#108562=AXIS2_PLACEMENT_3D('',#245533,#135195,#135196);
#108563=AXIS2_PLACEMENT_3D('',#245534,#135197,#135198);
#108564=AXIS2_PLACEMENT_3D('',#245535,#135199,#135200);
#108565=AXIS2_PLACEMENT_3D('',#245536,#135201,#135202);
#108566=AXIS2_PLACEMENT_3D('',#245537,#135203,#135204);
#108567=AXIS2_PLACEMENT_3D('',#245550,#135205,#135206);
#108568=AXIS2_PLACEMENT_3D('',#245551,#135207,#135208);
#108569=AXIS2_PLACEMENT_3D('',#245552,#135209,#135210);
#108570=AXIS2_PLACEMENT_3D('',#245553,#135211,#135212);
#108571=AXIS2_PLACEMENT_3D('',#245554,#135213,#135214);
#108572=AXIS2_PLACEMENT_3D('',#245567,#135215,#135216);
#108573=AXIS2_PLACEMENT_3D('',#245568,#135217,#135218);
#108574=AXIS2_PLACEMENT_3D('',#245569,#135219,#135220);
#108575=AXIS2_PLACEMENT_3D('',#245570,#135221,#135222);
#108576=AXIS2_PLACEMENT_3D('',#245571,#135223,#135224);
#108577=AXIS2_PLACEMENT_3D('',#245584,#135225,#135226);
#108578=AXIS2_PLACEMENT_3D('',#245597,#135227,#135228);
#108579=AXIS2_PLACEMENT_3D('',#245598,#135229,#135230);
#108580=AXIS2_PLACEMENT_3D('',#245599,#135231,#135232);
#108581=AXIS2_PLACEMENT_3D('',#245600,#135233,#135234);
#108582=AXIS2_PLACEMENT_3D('',#245601,#135235,#135236);
#108583=AXIS2_PLACEMENT_3D('',#245620,#135237,#135238);
#108584=AXIS2_PLACEMENT_3D('',#245621,#135239,#135240);
#108585=AXIS2_PLACEMENT_3D('',#245622,#135241,#135242);
#108586=AXIS2_PLACEMENT_3D('',#245623,#135243,#135244);
#108587=AXIS2_PLACEMENT_3D('',#245624,#135245,#135246);
#108588=AXIS2_PLACEMENT_3D('',#245637,#135247,#135248);
#108589=AXIS2_PLACEMENT_3D('',#245656,#135249,#135250);
#108590=AXIS2_PLACEMENT_3D('',#245657,#135251,#135252);
#108591=AXIS2_PLACEMENT_3D('',#245658,#135253,#135254);
#108592=AXIS2_PLACEMENT_3D('',#245659,#135255,#135256);
#108593=AXIS2_PLACEMENT_3D('',#245660,#135257,#135258);
#108594=AXIS2_PLACEMENT_3D('',#245679,#135259,#135260);
#108595=AXIS2_PLACEMENT_3D('',#245692,#135261,#135262);
#108596=AXIS2_PLACEMENT_3D('',#245693,#135263,#135264);
#108597=AXIS2_PLACEMENT_3D('',#245694,#135265,#135266);
#108598=AXIS2_PLACEMENT_3D('',#245695,#135267,#135268);
#108599=AXIS2_PLACEMENT_3D('',#245696,#135269,#135270);
#108600=AXIS2_PLACEMENT_3D('',#245715,#135271,#135272);
#108601=AXIS2_PLACEMENT_3D('',#245716,#135273,#135274);
#108602=AXIS2_PLACEMENT_3D('',#245717,#135275,#135276);
#108603=AXIS2_PLACEMENT_3D('',#245718,#135277,#135278);
#108604=AXIS2_PLACEMENT_3D('',#245719,#135279,#135280);
#108605=AXIS2_PLACEMENT_3D('',#245732,#135281,#135282);
#108606=AXIS2_PLACEMENT_3D('',#245745,#135283,#135284);
#108607=AXIS2_PLACEMENT_3D('',#245746,#135285,#135286);
#108608=AXIS2_PLACEMENT_3D('',#245747,#135287,#135288);
#108609=AXIS2_PLACEMENT_3D('',#245748,#135289,#135290);
#108610=AXIS2_PLACEMENT_3D('',#245749,#135291,#135292);
#108611=AXIS2_PLACEMENT_3D('',#245762,#135293,#135294);
#108612=AXIS2_PLACEMENT_3D('',#245763,#135295,#135296);
#108613=AXIS2_PLACEMENT_3D('',#245764,#135297,#135298);
#108614=AXIS2_PLACEMENT_3D('',#245765,#135299,#135300);
#108615=AXIS2_PLACEMENT_3D('',#245766,#135301,#135302);
#108616=AXIS2_PLACEMENT_3D('',#245779,#135303,#135304);
#108617=AXIS2_PLACEMENT_3D('',#245780,#135305,#135306);
#108618=AXIS2_PLACEMENT_3D('',#245781,#135307,#135308);
#108619=AXIS2_PLACEMENT_3D('',#245782,#135309,#135310);
#108620=AXIS2_PLACEMENT_3D('',#245783,#135311,#135312);
#108621=AXIS2_PLACEMENT_3D('',#245796,#135313,#135314);
#108622=AXIS2_PLACEMENT_3D('',#245809,#135315,#135316);
#108623=AXIS2_PLACEMENT_3D('',#245810,#135317,#135318);
#108624=AXIS2_PLACEMENT_3D('',#245811,#135319,#135320);
#108625=AXIS2_PLACEMENT_3D('',#245812,#135321,#135322);
#108626=AXIS2_PLACEMENT_3D('',#245813,#135323,#135324);
#108627=AXIS2_PLACEMENT_3D('',#245832,#135325,#135326);
#108628=AXIS2_PLACEMENT_3D('',#245833,#135327,#135328);
#108629=AXIS2_PLACEMENT_3D('',#245834,#135329,#135330);
#108630=AXIS2_PLACEMENT_3D('',#245835,#135331,#135332);
#108631=AXIS2_PLACEMENT_3D('',#245836,#135333,#135334);
#108632=AXIS2_PLACEMENT_3D('',#245849,#135335,#135336);
#108633=AXIS2_PLACEMENT_3D('',#245868,#135337,#135338);
#108634=AXIS2_PLACEMENT_3D('',#245869,#135339,#135340);
#108635=AXIS2_PLACEMENT_3D('',#245870,#135341,#135342);
#108636=AXIS2_PLACEMENT_3D('',#245871,#135343,#135344);
#108637=AXIS2_PLACEMENT_3D('',#245872,#135345,#135346);
#108638=AXIS2_PLACEMENT_3D('',#245891,#135347,#135348);
#108639=AXIS2_PLACEMENT_3D('',#245904,#135349,#135350);
#108640=AXIS2_PLACEMENT_3D('',#245905,#135351,#135352);
#108641=AXIS2_PLACEMENT_3D('',#245906,#135353,#135354);
#108642=AXIS2_PLACEMENT_3D('',#245907,#135355,#135356);
#108643=AXIS2_PLACEMENT_3D('',#245908,#135357,#135358);
#108644=AXIS2_PLACEMENT_3D('',#245927,#135359,#135360);
#108645=AXIS2_PLACEMENT_3D('',#245928,#135361,#135362);
#108646=AXIS2_PLACEMENT_3D('',#245929,#135363,#135364);
#108647=AXIS2_PLACEMENT_3D('',#245930,#135365,#135366);
#108648=AXIS2_PLACEMENT_3D('',#245931,#135367,#135368);
#108649=AXIS2_PLACEMENT_3D('',#245944,#135369,#135370);
#108650=AXIS2_PLACEMENT_3D('',#245957,#135371,#135372);
#108651=AXIS2_PLACEMENT_3D('',#245958,#135373,#135374);
#108652=AXIS2_PLACEMENT_3D('',#245959,#135375,#135376);
#108653=AXIS2_PLACEMENT_3D('',#245960,#135377,#135378);
#108654=AXIS2_PLACEMENT_3D('',#245961,#135379,#135380);
#108655=AXIS2_PLACEMENT_3D('',#245974,#135381,#135382);
#108656=AXIS2_PLACEMENT_3D('',#245975,#135383,#135384);
#108657=AXIS2_PLACEMENT_3D('',#245976,#135385,#135386);
#108658=AXIS2_PLACEMENT_3D('',#245977,#135387,#135388);
#108659=AXIS2_PLACEMENT_3D('',#245978,#135389,#135390);
#108660=AXIS2_PLACEMENT_3D('',#245991,#135391,#135392);
#108661=AXIS2_PLACEMENT_3D('',#245992,#135393,#135394);
#108662=AXIS2_PLACEMENT_3D('',#245993,#135395,#135396);
#108663=AXIS2_PLACEMENT_3D('',#245994,#135397,#135398);
#108664=AXIS2_PLACEMENT_3D('',#245995,#135399,#135400);
#108665=AXIS2_PLACEMENT_3D('',#246008,#135401,#135402);
#108666=AXIS2_PLACEMENT_3D('',#246021,#135403,#135404);
#108667=AXIS2_PLACEMENT_3D('',#246022,#135405,#135406);
#108668=AXIS2_PLACEMENT_3D('',#246023,#135407,#135408);
#108669=AXIS2_PLACEMENT_3D('',#246024,#135409,#135410);
#108670=AXIS2_PLACEMENT_3D('',#246025,#135411,#135412);
#108671=AXIS2_PLACEMENT_3D('',#246044,#135413,#135414);
#108672=AXIS2_PLACEMENT_3D('',#246045,#135415,#135416);
#108673=AXIS2_PLACEMENT_3D('',#246046,#135417,#135418);
#108674=AXIS2_PLACEMENT_3D('',#246047,#135419,#135420);
#108675=AXIS2_PLACEMENT_3D('',#246048,#135421,#135422);
#108676=AXIS2_PLACEMENT_3D('',#246061,#135423,#135424);
#108677=AXIS2_PLACEMENT_3D('',#246080,#135425,#135426);
#108678=AXIS2_PLACEMENT_3D('',#246081,#135427,#135428);
#108679=AXIS2_PLACEMENT_3D('',#246082,#135429,#135430);
#108680=AXIS2_PLACEMENT_3D('',#246083,#135431,#135432);
#108681=AXIS2_PLACEMENT_3D('',#246084,#135433,#135434);
#108682=AXIS2_PLACEMENT_3D('',#246103,#135435,#135436);
#108683=AXIS2_PLACEMENT_3D('',#246116,#135437,#135438);
#108684=AXIS2_PLACEMENT_3D('',#246117,#135439,#135440);
#108685=AXIS2_PLACEMENT_3D('',#246118,#135441,#135442);
#108686=AXIS2_PLACEMENT_3D('',#246119,#135443,#135444);
#108687=AXIS2_PLACEMENT_3D('',#246120,#135445,#135446);
#108688=AXIS2_PLACEMENT_3D('',#246139,#135447,#135448);
#108689=AXIS2_PLACEMENT_3D('',#246140,#135449,#135450);
#108690=AXIS2_PLACEMENT_3D('',#246141,#135451,#135452);
#108691=AXIS2_PLACEMENT_3D('',#246142,#135453,#135454);
#108692=AXIS2_PLACEMENT_3D('',#246143,#135455,#135456);
#108693=AXIS2_PLACEMENT_3D('',#246156,#135457,#135458);
#108694=AXIS2_PLACEMENT_3D('',#246169,#135459,#135460);
#108695=AXIS2_PLACEMENT_3D('',#246170,#135461,#135462);
#108696=AXIS2_PLACEMENT_3D('',#246171,#135463,#135464);
#108697=AXIS2_PLACEMENT_3D('',#246172,#135465,#135466);
#108698=AXIS2_PLACEMENT_3D('',#246173,#135467,#135468);
#108699=AXIS2_PLACEMENT_3D('',#246186,#135469,#135470);
#108700=AXIS2_PLACEMENT_3D('',#246187,#135471,#135472);
#108701=AXIS2_PLACEMENT_3D('',#246188,#135473,#135474);
#108702=AXIS2_PLACEMENT_3D('',#246189,#135475,#135476);
#108703=AXIS2_PLACEMENT_3D('',#246190,#135477,#135478);
#108704=AXIS2_PLACEMENT_3D('',#246203,#135479,#135480);
#108705=AXIS2_PLACEMENT_3D('',#246204,#135481,#135482);
#108706=AXIS2_PLACEMENT_3D('',#246205,#135483,#135484);
#108707=AXIS2_PLACEMENT_3D('',#246206,#135485,#135486);
#108708=AXIS2_PLACEMENT_3D('',#246207,#135487,#135488);
#108709=AXIS2_PLACEMENT_3D('',#246220,#135489,#135490);
#108710=AXIS2_PLACEMENT_3D('',#246233,#135491,#135492);
#108711=AXIS2_PLACEMENT_3D('',#246234,#135493,#135494);
#108712=AXIS2_PLACEMENT_3D('',#246235,#135495,#135496);
#108713=AXIS2_PLACEMENT_3D('',#246236,#135497,#135498);
#108714=AXIS2_PLACEMENT_3D('',#246237,#135499,#135500);
#108715=AXIS2_PLACEMENT_3D('',#246256,#135501,#135502);
#108716=AXIS2_PLACEMENT_3D('',#246257,#135503,#135504);
#108717=AXIS2_PLACEMENT_3D('',#246258,#135505,#135506);
#108718=AXIS2_PLACEMENT_3D('',#246259,#135507,#135508);
#108719=AXIS2_PLACEMENT_3D('',#246260,#135509,#135510);
#108720=AXIS2_PLACEMENT_3D('',#246273,#135511,#135512);
#108721=AXIS2_PLACEMENT_3D('',#246292,#135513,#135514);
#108722=AXIS2_PLACEMENT_3D('',#246293,#135515,#135516);
#108723=AXIS2_PLACEMENT_3D('',#246294,#135517,#135518);
#108724=AXIS2_PLACEMENT_3D('',#246295,#135519,#135520);
#108725=AXIS2_PLACEMENT_3D('',#246296,#135521,#135522);
#108726=AXIS2_PLACEMENT_3D('',#246315,#135523,#135524);
#108727=AXIS2_PLACEMENT_3D('',#246328,#135525,#135526);
#108728=AXIS2_PLACEMENT_3D('',#246329,#135527,#135528);
#108729=AXIS2_PLACEMENT_3D('',#246330,#135529,#135530);
#108730=AXIS2_PLACEMENT_3D('',#246331,#135531,#135532);
#108731=AXIS2_PLACEMENT_3D('',#246332,#135533,#135534);
#108732=AXIS2_PLACEMENT_3D('',#246351,#135535,#135536);
#108733=AXIS2_PLACEMENT_3D('',#246352,#135537,#135538);
#108734=AXIS2_PLACEMENT_3D('',#246353,#135539,#135540);
#108735=AXIS2_PLACEMENT_3D('',#246354,#135541,#135542);
#108736=AXIS2_PLACEMENT_3D('',#246355,#135543,#135544);
#108737=AXIS2_PLACEMENT_3D('',#246368,#135545,#135546);
#108738=AXIS2_PLACEMENT_3D('',#246381,#135547,#135548);
#108739=AXIS2_PLACEMENT_3D('',#246382,#135549,#135550);
#108740=AXIS2_PLACEMENT_3D('',#246383,#135551,#135552);
#108741=AXIS2_PLACEMENT_3D('',#246384,#135553,#135554);
#108742=AXIS2_PLACEMENT_3D('',#246385,#135555,#135556);
#108743=AXIS2_PLACEMENT_3D('',#246398,#135557,#135558);
#108744=AXIS2_PLACEMENT_3D('',#246399,#135559,#135560);
#108745=AXIS2_PLACEMENT_3D('',#246400,#135561,#135562);
#108746=AXIS2_PLACEMENT_3D('',#246401,#135563,#135564);
#108747=AXIS2_PLACEMENT_3D('',#246402,#135565,#135566);
#108748=AXIS2_PLACEMENT_3D('',#246415,#135567,#135568);
#108749=AXIS2_PLACEMENT_3D('',#246416,#135569,#135570);
#108750=AXIS2_PLACEMENT_3D('',#246417,#135571,#135572);
#108751=AXIS2_PLACEMENT_3D('',#246418,#135573,#135574);
#108752=AXIS2_PLACEMENT_3D('',#246419,#135575,#135576);
#108753=AXIS2_PLACEMENT_3D('',#246432,#135577,#135578);
#108754=AXIS2_PLACEMENT_3D('',#246445,#135579,#135580);
#108755=AXIS2_PLACEMENT_3D('',#246446,#135581,#135582);
#108756=AXIS2_PLACEMENT_3D('',#246447,#135583,#135584);
#108757=AXIS2_PLACEMENT_3D('',#246448,#135585,#135586);
#108758=AXIS2_PLACEMENT_3D('',#246449,#135587,#135588);
#108759=AXIS2_PLACEMENT_3D('',#246468,#135589,#135590);
#108760=AXIS2_PLACEMENT_3D('',#246469,#135591,#135592);
#108761=AXIS2_PLACEMENT_3D('',#246470,#135593,#135594);
#108762=AXIS2_PLACEMENT_3D('',#246471,#135595,#135596);
#108763=AXIS2_PLACEMENT_3D('',#246472,#135597,#135598);
#108764=AXIS2_PLACEMENT_3D('',#246485,#135599,#135600);
#108765=AXIS2_PLACEMENT_3D('',#246504,#135601,#135602);
#108766=AXIS2_PLACEMENT_3D('',#246505,#135603,#135604);
#108767=AXIS2_PLACEMENT_3D('',#246506,#135605,#135606);
#108768=AXIS2_PLACEMENT_3D('',#246507,#135607,#135608);
#108769=AXIS2_PLACEMENT_3D('',#246508,#135609,#135610);
#108770=AXIS2_PLACEMENT_3D('',#246527,#135611,#135612);
#108771=AXIS2_PLACEMENT_3D('',#246540,#135613,#135614);
#108772=AXIS2_PLACEMENT_3D('',#246541,#135615,#135616);
#108773=AXIS2_PLACEMENT_3D('',#246542,#135617,#135618);
#108774=AXIS2_PLACEMENT_3D('',#246543,#135619,#135620);
#108775=AXIS2_PLACEMENT_3D('',#246544,#135621,#135622);
#108776=AXIS2_PLACEMENT_3D('',#246563,#135623,#135624);
#108777=AXIS2_PLACEMENT_3D('',#246564,#135625,#135626);
#108778=AXIS2_PLACEMENT_3D('',#246565,#135627,#135628);
#108779=AXIS2_PLACEMENT_3D('',#246566,#135629,#135630);
#108780=AXIS2_PLACEMENT_3D('',#246567,#135631,#135632);
#108781=AXIS2_PLACEMENT_3D('',#246580,#135633,#135634);
#108782=AXIS2_PLACEMENT_3D('',#246593,#135635,#135636);
#108783=AXIS2_PLACEMENT_3D('',#246594,#135637,#135638);
#108784=AXIS2_PLACEMENT_3D('',#246595,#135639,#135640);
#108785=AXIS2_PLACEMENT_3D('',#246596,#135641,#135642);
#108786=AXIS2_PLACEMENT_3D('',#246597,#135643,#135644);
#108787=AXIS2_PLACEMENT_3D('',#246610,#135645,#135646);
#108788=AXIS2_PLACEMENT_3D('',#246611,#135647,#135648);
#108789=AXIS2_PLACEMENT_3D('',#246612,#135649,#135650);
#108790=AXIS2_PLACEMENT_3D('',#246613,#135651,#135652);
#108791=AXIS2_PLACEMENT_3D('',#246614,#135653,#135654);
#108792=AXIS2_PLACEMENT_3D('',#246627,#135655,#135656);
#108793=AXIS2_PLACEMENT_3D('',#246628,#135657,#135658);
#108794=AXIS2_PLACEMENT_3D('',#246629,#135659,#135660);
#108795=AXIS2_PLACEMENT_3D('',#246630,#135661,#135662);
#108796=AXIS2_PLACEMENT_3D('',#246631,#135663,#135664);
#108797=AXIS2_PLACEMENT_3D('',#246644,#135665,#135666);
#108798=AXIS2_PLACEMENT_3D('',#246657,#135667,#135668);
#108799=AXIS2_PLACEMENT_3D('',#246658,#135669,#135670);
#108800=AXIS2_PLACEMENT_3D('',#246659,#135671,#135672);
#108801=AXIS2_PLACEMENT_3D('',#246660,#135673,#135674);
#108802=AXIS2_PLACEMENT_3D('',#246661,#135675,#135676);
#108803=AXIS2_PLACEMENT_3D('',#246680,#135677,#135678);
#108804=AXIS2_PLACEMENT_3D('',#246681,#135679,#135680);
#108805=AXIS2_PLACEMENT_3D('',#246682,#135681,#135682);
#108806=AXIS2_PLACEMENT_3D('',#246683,#135683,#135684);
#108807=AXIS2_PLACEMENT_3D('',#246684,#135685,#135686);
#108808=AXIS2_PLACEMENT_3D('',#246697,#135687,#135688);
#108809=AXIS2_PLACEMENT_3D('',#246716,#135689,#135690);
#108810=AXIS2_PLACEMENT_3D('',#246717,#135691,#135692);
#108811=AXIS2_PLACEMENT_3D('',#246718,#135693,#135694);
#108812=AXIS2_PLACEMENT_3D('',#246719,#135695,#135696);
#108813=AXIS2_PLACEMENT_3D('',#246720,#135697,#135698);
#108814=AXIS2_PLACEMENT_3D('',#246739,#135699,#135700);
#108815=AXIS2_PLACEMENT_3D('',#246752,#135701,#135702);
#108816=AXIS2_PLACEMENT_3D('',#246753,#135703,#135704);
#108817=AXIS2_PLACEMENT_3D('',#246754,#135705,#135706);
#108818=AXIS2_PLACEMENT_3D('',#246755,#135707,#135708);
#108819=AXIS2_PLACEMENT_3D('',#246756,#135709,#135710);
#108820=AXIS2_PLACEMENT_3D('',#246775,#135711,#135712);
#108821=AXIS2_PLACEMENT_3D('',#246776,#135713,#135714);
#108822=AXIS2_PLACEMENT_3D('',#246777,#135715,#135716);
#108823=AXIS2_PLACEMENT_3D('',#246778,#135717,#135718);
#108824=AXIS2_PLACEMENT_3D('',#246779,#135719,#135720);
#108825=AXIS2_PLACEMENT_3D('',#246792,#135721,#135722);
#108826=AXIS2_PLACEMENT_3D('',#246805,#135723,#135724);
#108827=AXIS2_PLACEMENT_3D('',#246806,#135725,#135726);
#108828=AXIS2_PLACEMENT_3D('',#246807,#135727,#135728);
#108829=AXIS2_PLACEMENT_3D('',#246808,#135729,#135730);
#108830=AXIS2_PLACEMENT_3D('',#246809,#135731,#135732);
#108831=AXIS2_PLACEMENT_3D('',#246822,#135733,#135734);
#108832=AXIS2_PLACEMENT_3D('',#246823,#135735,#135736);
#108833=AXIS2_PLACEMENT_3D('',#246824,#135737,#135738);
#108834=AXIS2_PLACEMENT_3D('',#246825,#135739,#135740);
#108835=AXIS2_PLACEMENT_3D('',#246826,#135741,#135742);
#108836=AXIS2_PLACEMENT_3D('',#246839,#135743,#135744);
#108837=AXIS2_PLACEMENT_3D('',#246840,#135745,#135746);
#108838=AXIS2_PLACEMENT_3D('',#246841,#135747,#135748);
#108839=AXIS2_PLACEMENT_3D('',#246842,#135749,#135750);
#108840=AXIS2_PLACEMENT_3D('',#246843,#135751,#135752);
#108841=AXIS2_PLACEMENT_3D('',#246856,#135753,#135754);
#108842=AXIS2_PLACEMENT_3D('',#246869,#135755,#135756);
#108843=AXIS2_PLACEMENT_3D('',#246870,#135757,#135758);
#108844=AXIS2_PLACEMENT_3D('',#246871,#135759,#135760);
#108845=AXIS2_PLACEMENT_3D('',#246872,#135761,#135762);
#108846=AXIS2_PLACEMENT_3D('',#246873,#135763,#135764);
#108847=AXIS2_PLACEMENT_3D('',#246892,#135765,#135766);
#108848=AXIS2_PLACEMENT_3D('',#246893,#135767,#135768);
#108849=AXIS2_PLACEMENT_3D('',#246894,#135769,#135770);
#108850=AXIS2_PLACEMENT_3D('',#246895,#135771,#135772);
#108851=AXIS2_PLACEMENT_3D('',#246896,#135773,#135774);
#108852=AXIS2_PLACEMENT_3D('',#246909,#135775,#135776);
#108853=AXIS2_PLACEMENT_3D('',#246928,#135777,#135778);
#108854=AXIS2_PLACEMENT_3D('',#246929,#135779,#135780);
#108855=AXIS2_PLACEMENT_3D('',#246930,#135781,#135782);
#108856=AXIS2_PLACEMENT_3D('',#246931,#135783,#135784);
#108857=AXIS2_PLACEMENT_3D('',#246932,#135785,#135786);
#108858=AXIS2_PLACEMENT_3D('',#246951,#135787,#135788);
#108859=AXIS2_PLACEMENT_3D('',#246964,#135789,#135790);
#108860=AXIS2_PLACEMENT_3D('',#246965,#135791,#135792);
#108861=AXIS2_PLACEMENT_3D('',#246966,#135793,#135794);
#108862=AXIS2_PLACEMENT_3D('',#246967,#135795,#135796);
#108863=AXIS2_PLACEMENT_3D('',#246968,#135797,#135798);
#108864=AXIS2_PLACEMENT_3D('',#246987,#135799,#135800);
#108865=AXIS2_PLACEMENT_3D('',#246988,#135801,#135802);
#108866=AXIS2_PLACEMENT_3D('',#246989,#135803,#135804);
#108867=AXIS2_PLACEMENT_3D('',#246990,#135805,#135806);
#108868=AXIS2_PLACEMENT_3D('',#246991,#135807,#135808);
#108869=AXIS2_PLACEMENT_3D('',#247004,#135809,#135810);
#108870=AXIS2_PLACEMENT_3D('',#247017,#135811,#135812);
#108871=AXIS2_PLACEMENT_3D('',#247018,#135813,#135814);
#108872=AXIS2_PLACEMENT_3D('',#247019,#135815,#135816);
#108873=AXIS2_PLACEMENT_3D('',#247020,#135817,#135818);
#108874=AXIS2_PLACEMENT_3D('',#247021,#135819,#135820);
#108875=AXIS2_PLACEMENT_3D('',#247034,#135821,#135822);
#108876=AXIS2_PLACEMENT_3D('',#247035,#135823,#135824);
#108877=AXIS2_PLACEMENT_3D('',#247036,#135825,#135826);
#108878=AXIS2_PLACEMENT_3D('',#247037,#135827,#135828);
#108879=AXIS2_PLACEMENT_3D('',#247038,#135829,#135830);
#108880=AXIS2_PLACEMENT_3D('',#247051,#135831,#135832);
#108881=AXIS2_PLACEMENT_3D('',#247052,#135833,#135834);
#108882=AXIS2_PLACEMENT_3D('',#247053,#135835,#135836);
#108883=AXIS2_PLACEMENT_3D('',#247054,#135837,#135838);
#108884=AXIS2_PLACEMENT_3D('',#247055,#135839,#135840);
#108885=AXIS2_PLACEMENT_3D('',#247068,#135841,#135842);
#108886=AXIS2_PLACEMENT_3D('',#247081,#135843,#135844);
#108887=AXIS2_PLACEMENT_3D('',#247082,#135845,#135846);
#108888=AXIS2_PLACEMENT_3D('',#247083,#135847,#135848);
#108889=AXIS2_PLACEMENT_3D('',#247084,#135849,#135850);
#108890=AXIS2_PLACEMENT_3D('',#247085,#135851,#135852);
#108891=AXIS2_PLACEMENT_3D('',#247104,#135853,#135854);
#108892=AXIS2_PLACEMENT_3D('',#247105,#135855,#135856);
#108893=AXIS2_PLACEMENT_3D('',#247118,#135857,#135858);
#108894=AXIS2_PLACEMENT_3D('',#247137,#135859,#135860);
#108895=AXIS2_PLACEMENT_3D('',#247138,#135861,#135862);
#108896=AXIS2_PLACEMENT_3D('',#247139,#135863,#135864);
#108897=AXIS2_PLACEMENT_3D('',#247140,#135865,#135866);
#108898=AXIS2_PLACEMENT_3D('',#247141,#135867,#135868);
#108899=AXIS2_PLACEMENT_3D('',#247172,#135869,#135870);
#108900=AXIS2_PLACEMENT_3D('',#247173,#135871,#135872);
#108901=AXIS2_PLACEMENT_3D('',#247174,#135873,#135874);
#108902=AXIS2_PLACEMENT_3D('',#247193,#135875,#135876);
#108903=AXIS2_PLACEMENT_3D('',#247194,#135877,#135878);
#108904=AXIS2_PLACEMENT_3D('',#247195,#135879,#135880);
#108905=AXIS2_PLACEMENT_3D('',#247196,#135881,#135882);
#108906=AXIS2_PLACEMENT_3D('',#247197,#135883,#135884);
#108907=AXIS2_PLACEMENT_3D('',#247210,#135885,#135886);
#108908=AXIS2_PLACEMENT_3D('',#247223,#135887,#135888);
#108909=AXIS2_PLACEMENT_3D('',#247224,#135889,#135890);
#108910=AXIS2_PLACEMENT_3D('',#247225,#135891,#135892);
#108911=AXIS2_PLACEMENT_3D('',#247226,#135893,#135894);
#108912=AXIS2_PLACEMENT_3D('',#247227,#135895,#135896);
#108913=AXIS2_PLACEMENT_3D('',#247240,#135897,#135898);
#108914=AXIS2_PLACEMENT_3D('',#247241,#135899,#135900);
#108915=AXIS2_PLACEMENT_3D('',#247242,#135901,#135902);
#108916=AXIS2_PLACEMENT_3D('',#247243,#135903,#135904);
#108917=AXIS2_PLACEMENT_3D('',#247244,#135905,#135906);
#108918=AXIS2_PLACEMENT_3D('',#247257,#135907,#135908);
#108919=AXIS2_PLACEMENT_3D('',#247258,#135909,#135910);
#108920=AXIS2_PLACEMENT_3D('',#247259,#135911,#135912);
#108921=AXIS2_PLACEMENT_3D('',#247260,#135913,#135914);
#108922=AXIS2_PLACEMENT_3D('',#247261,#135915,#135916);
#108923=AXIS2_PLACEMENT_3D('',#247274,#135917,#135918);
#108924=AXIS2_PLACEMENT_3D('',#247287,#135919,#135920);
#108925=AXIS2_PLACEMENT_3D('',#247288,#135921,#135922);
#108926=AXIS2_PLACEMENT_3D('',#247289,#135923,#135924);
#108927=AXIS2_PLACEMENT_3D('',#247290,#135925,#135926);
#108928=AXIS2_PLACEMENT_3D('',#247291,#135927,#135928);
#108929=AXIS2_PLACEMENT_3D('',#247310,#135929,#135930);
#108930=AXIS2_PLACEMENT_3D('',#247311,#135931,#135932);
#108931=AXIS2_PLACEMENT_3D('',#247312,#135933,#135934);
#108932=AXIS2_PLACEMENT_3D('',#247313,#135935,#135936);
#108933=AXIS2_PLACEMENT_3D('',#247314,#135937,#135938);
#108934=AXIS2_PLACEMENT_3D('',#247327,#135939,#135940);
#108935=AXIS2_PLACEMENT_3D('',#247346,#135941,#135942);
#108936=AXIS2_PLACEMENT_3D('',#247347,#135943,#135944);
#108937=AXIS2_PLACEMENT_3D('',#247348,#135945,#135946);
#108938=AXIS2_PLACEMENT_3D('',#247349,#135947,#135948);
#108939=AXIS2_PLACEMENT_3D('',#247350,#135949,#135950);
#108940=AXIS2_PLACEMENT_3D('',#247369,#135951,#135952);
#108941=AXIS2_PLACEMENT_3D('',#247382,#135953,#135954);
#108942=AXIS2_PLACEMENT_3D('',#247383,#135955,#135956);
#108943=AXIS2_PLACEMENT_3D('',#247384,#135957,#135958);
#108944=AXIS2_PLACEMENT_3D('',#247385,#135959,#135960);
#108945=AXIS2_PLACEMENT_3D('',#247386,#135961,#135962);
#108946=AXIS2_PLACEMENT_3D('',#247405,#135963,#135964);
#108947=AXIS2_PLACEMENT_3D('',#247406,#135965,#135966);
#108948=AXIS2_PLACEMENT_3D('',#247407,#135967,#135968);
#108949=AXIS2_PLACEMENT_3D('',#247408,#135969,#135970);
#108950=AXIS2_PLACEMENT_3D('',#247409,#135971,#135972);
#108951=AXIS2_PLACEMENT_3D('',#247422,#135973,#135974);
#108952=AXIS2_PLACEMENT_3D('',#247435,#135975,#135976);
#108953=AXIS2_PLACEMENT_3D('',#247436,#135977,#135978);
#108954=AXIS2_PLACEMENT_3D('',#247437,#135979,#135980);
#108955=AXIS2_PLACEMENT_3D('',#247438,#135981,#135982);
#108956=AXIS2_PLACEMENT_3D('',#247439,#135983,#135984);
#108957=AXIS2_PLACEMENT_3D('',#247452,#135985,#135986);
#108958=AXIS2_PLACEMENT_3D('',#247453,#135987,#135988);
#108959=AXIS2_PLACEMENT_3D('',#247454,#135989,#135990);
#108960=AXIS2_PLACEMENT_3D('',#247455,#135991,#135992);
#108961=AXIS2_PLACEMENT_3D('',#247456,#135993,#135994);
#108962=AXIS2_PLACEMENT_3D('',#247469,#135995,#135996);
#108963=AXIS2_PLACEMENT_3D('',#247470,#135997,#135998);
#108964=AXIS2_PLACEMENT_3D('',#247471,#135999,#136000);
#108965=AXIS2_PLACEMENT_3D('',#247472,#136001,#136002);
#108966=AXIS2_PLACEMENT_3D('',#247473,#136003,#136004);
#108967=AXIS2_PLACEMENT_3D('',#247486,#136005,#136006);
#108968=AXIS2_PLACEMENT_3D('',#247499,#136007,#136008);
#108969=AXIS2_PLACEMENT_3D('',#247500,#136009,#136010);
#108970=AXIS2_PLACEMENT_3D('',#247501,#136011,#136012);
#108971=AXIS2_PLACEMENT_3D('',#247502,#136013,#136014);
#108972=AXIS2_PLACEMENT_3D('',#247503,#136015,#136016);
#108973=AXIS2_PLACEMENT_3D('',#247522,#136017,#136018);
#108974=AXIS2_PLACEMENT_3D('',#247523,#136019,#136020);
#108975=AXIS2_PLACEMENT_3D('',#247524,#136021,#136022);
#108976=AXIS2_PLACEMENT_3D('',#247525,#136023,#136024);
#108977=AXIS2_PLACEMENT_3D('',#247526,#136025,#136026);
#108978=AXIS2_PLACEMENT_3D('',#247539,#136027,#136028);
#108979=AXIS2_PLACEMENT_3D('',#247558,#136029,#136030);
#108980=AXIS2_PLACEMENT_3D('',#247559,#136031,#136032);
#108981=AXIS2_PLACEMENT_3D('',#247560,#136033,#136034);
#108982=AXIS2_PLACEMENT_3D('',#247561,#136035,#136036);
#108983=AXIS2_PLACEMENT_3D('',#247562,#136037,#136038);
#108984=AXIS2_PLACEMENT_3D('',#247581,#136039,#136040);
#108985=AXIS2_PLACEMENT_3D('',#247594,#136041,#136042);
#108986=AXIS2_PLACEMENT_3D('',#247595,#136043,#136044);
#108987=AXIS2_PLACEMENT_3D('',#247596,#136045,#136046);
#108988=AXIS2_PLACEMENT_3D('',#247597,#136047,#136048);
#108989=AXIS2_PLACEMENT_3D('',#247598,#136049,#136050);
#108990=AXIS2_PLACEMENT_3D('',#247617,#136051,#136052);
#108991=AXIS2_PLACEMENT_3D('',#247618,#136053,#136054);
#108992=AXIS2_PLACEMENT_3D('',#247619,#136055,#136056);
#108993=AXIS2_PLACEMENT_3D('',#247620,#136057,#136058);
#108994=AXIS2_PLACEMENT_3D('',#247621,#136059,#136060);
#108995=AXIS2_PLACEMENT_3D('',#247634,#136061,#136062);
#108996=AXIS2_PLACEMENT_3D('',#247647,#136063,#136064);
#108997=AXIS2_PLACEMENT_3D('',#247648,#136065,#136066);
#108998=AXIS2_PLACEMENT_3D('',#247649,#136067,#136068);
#108999=AXIS2_PLACEMENT_3D('',#247650,#136069,#136070);
#109000=AXIS2_PLACEMENT_3D('',#247651,#136071,#136072);
#109001=AXIS2_PLACEMENT_3D('',#247664,#136073,#136074);
#109002=AXIS2_PLACEMENT_3D('',#247665,#136075,#136076);
#109003=AXIS2_PLACEMENT_3D('',#247666,#136077,#136078);
#109004=AXIS2_PLACEMENT_3D('',#247667,#136079,#136080);
#109005=AXIS2_PLACEMENT_3D('',#247668,#136081,#136082);
#109006=AXIS2_PLACEMENT_3D('',#247681,#136083,#136084);
#109007=AXIS2_PLACEMENT_3D('',#247682,#136085,#136086);
#109008=AXIS2_PLACEMENT_3D('',#247683,#136087,#136088);
#109009=AXIS2_PLACEMENT_3D('',#247684,#136089,#136090);
#109010=AXIS2_PLACEMENT_3D('',#247685,#136091,#136092);
#109011=AXIS2_PLACEMENT_3D('',#247698,#136093,#136094);
#109012=AXIS2_PLACEMENT_3D('',#247711,#136095,#136096);
#109013=AXIS2_PLACEMENT_3D('',#247712,#136097,#136098);
#109014=AXIS2_PLACEMENT_3D('',#247713,#136099,#136100);
#109015=AXIS2_PLACEMENT_3D('',#247714,#136101,#136102);
#109016=AXIS2_PLACEMENT_3D('',#247715,#136103,#136104);
#109017=AXIS2_PLACEMENT_3D('',#247734,#136105,#136106);
#109018=AXIS2_PLACEMENT_3D('',#247735,#136107,#136108);
#109019=AXIS2_PLACEMENT_3D('',#247736,#136109,#136110);
#109020=AXIS2_PLACEMENT_3D('',#247737,#136111,#136112);
#109021=AXIS2_PLACEMENT_3D('',#247738,#136113,#136114);
#109022=AXIS2_PLACEMENT_3D('',#247751,#136115,#136116);
#109023=AXIS2_PLACEMENT_3D('',#247770,#136117,#136118);
#109024=AXIS2_PLACEMENT_3D('',#247771,#136119,#136120);
#109025=AXIS2_PLACEMENT_3D('',#247772,#136121,#136122);
#109026=AXIS2_PLACEMENT_3D('',#247773,#136123,#136124);
#109027=AXIS2_PLACEMENT_3D('',#247774,#136125,#136126);
#109028=AXIS2_PLACEMENT_3D('',#247793,#136127,#136128);
#109029=AXIS2_PLACEMENT_3D('',#247806,#136129,#136130);
#109030=AXIS2_PLACEMENT_3D('',#247807,#136131,#136132);
#109031=AXIS2_PLACEMENT_3D('',#247808,#136133,#136134);
#109032=AXIS2_PLACEMENT_3D('',#247809,#136135,#136136);
#109033=AXIS2_PLACEMENT_3D('',#247810,#136137,#136138);
#109034=AXIS2_PLACEMENT_3D('',#247829,#136139,#136140);
#109035=AXIS2_PLACEMENT_3D('',#247830,#136141,#136142);
#109036=AXIS2_PLACEMENT_3D('',#247831,#136143,#136144);
#109037=AXIS2_PLACEMENT_3D('',#247832,#136145,#136146);
#109038=AXIS2_PLACEMENT_3D('',#247833,#136147,#136148);
#109039=AXIS2_PLACEMENT_3D('',#247846,#136149,#136150);
#109040=AXIS2_PLACEMENT_3D('',#247859,#136151,#136152);
#109041=AXIS2_PLACEMENT_3D('',#247860,#136153,#136154);
#109042=AXIS2_PLACEMENT_3D('',#247861,#136155,#136156);
#109043=AXIS2_PLACEMENT_3D('',#247862,#136157,#136158);
#109044=AXIS2_PLACEMENT_3D('',#247863,#136159,#136160);
#109045=AXIS2_PLACEMENT_3D('',#247876,#136161,#136162);
#109046=AXIS2_PLACEMENT_3D('',#247877,#136163,#136164);
#109047=AXIS2_PLACEMENT_3D('',#247878,#136165,#136166);
#109048=AXIS2_PLACEMENT_3D('',#247879,#136167,#136168);
#109049=AXIS2_PLACEMENT_3D('',#247880,#136169,#136170);
#109050=AXIS2_PLACEMENT_3D('',#247893,#136171,#136172);
#109051=AXIS2_PLACEMENT_3D('',#247894,#136173,#136174);
#109052=AXIS2_PLACEMENT_3D('',#247895,#136175,#136176);
#109053=AXIS2_PLACEMENT_3D('',#247896,#136177,#136178);
#109054=AXIS2_PLACEMENT_3D('',#247897,#136179,#136180);
#109055=AXIS2_PLACEMENT_3D('',#247910,#136181,#136182);
#109056=AXIS2_PLACEMENT_3D('',#247923,#136183,#136184);
#109057=AXIS2_PLACEMENT_3D('',#247924,#136185,#136186);
#109058=AXIS2_PLACEMENT_3D('',#247925,#136187,#136188);
#109059=AXIS2_PLACEMENT_3D('',#247926,#136189,#136190);
#109060=AXIS2_PLACEMENT_3D('',#247927,#136191,#136192);
#109061=AXIS2_PLACEMENT_3D('',#247946,#136193,#136194);
#109062=AXIS2_PLACEMENT_3D('',#247947,#136195,#136196);
#109063=AXIS2_PLACEMENT_3D('',#247948,#136197,#136198);
#109064=AXIS2_PLACEMENT_3D('',#247949,#136199,#136200);
#109065=AXIS2_PLACEMENT_3D('',#247950,#136201,#136202);
#109066=AXIS2_PLACEMENT_3D('',#247963,#136203,#136204);
#109067=AXIS2_PLACEMENT_3D('',#247982,#136205,#136206);
#109068=AXIS2_PLACEMENT_3D('',#247983,#136207,#136208);
#109069=AXIS2_PLACEMENT_3D('',#247984,#136209,#136210);
#109070=AXIS2_PLACEMENT_3D('',#247985,#136211,#136212);
#109071=AXIS2_PLACEMENT_3D('',#247986,#136213,#136214);
#109072=AXIS2_PLACEMENT_3D('',#248005,#136215,#136216);
#109073=AXIS2_PLACEMENT_3D('',#248018,#136217,#136218);
#109074=AXIS2_PLACEMENT_3D('',#248019,#136219,#136220);
#109075=AXIS2_PLACEMENT_3D('',#248020,#136221,#136222);
#109076=AXIS2_PLACEMENT_3D('',#248021,#136223,#136224);
#109077=AXIS2_PLACEMENT_3D('',#248022,#136225,#136226);
#109078=AXIS2_PLACEMENT_3D('',#248041,#136227,#136228);
#109079=AXIS2_PLACEMENT_3D('',#248042,#136229,#136230);
#109080=AXIS2_PLACEMENT_3D('',#248043,#136231,#136232);
#109081=AXIS2_PLACEMENT_3D('',#248044,#136233,#136234);
#109082=AXIS2_PLACEMENT_3D('',#248045,#136235,#136236);
#109083=AXIS2_PLACEMENT_3D('',#248058,#136237,#136238);
#109084=AXIS2_PLACEMENT_3D('',#248071,#136239,#136240);
#109085=AXIS2_PLACEMENT_3D('',#248072,#136241,#136242);
#109086=AXIS2_PLACEMENT_3D('',#248073,#136243,#136244);
#109087=AXIS2_PLACEMENT_3D('',#248074,#136245,#136246);
#109088=AXIS2_PLACEMENT_3D('',#248075,#136247,#136248);
#109089=AXIS2_PLACEMENT_3D('',#248088,#136249,#136250);
#109090=AXIS2_PLACEMENT_3D('',#248089,#136251,#136252);
#109091=AXIS2_PLACEMENT_3D('',#248090,#136253,#136254);
#109092=AXIS2_PLACEMENT_3D('',#248091,#136255,#136256);
#109093=AXIS2_PLACEMENT_3D('',#248092,#136257,#136258);
#109094=AXIS2_PLACEMENT_3D('',#248105,#136259,#136260);
#109095=AXIS2_PLACEMENT_3D('',#248106,#136261,#136262);
#109096=AXIS2_PLACEMENT_3D('',#248107,#136263,#136264);
#109097=AXIS2_PLACEMENT_3D('',#248108,#136265,#136266);
#109098=AXIS2_PLACEMENT_3D('',#248109,#136267,#136268);
#109099=AXIS2_PLACEMENT_3D('',#248122,#136269,#136270);
#109100=AXIS2_PLACEMENT_3D('',#248135,#136271,#136272);
#109101=AXIS2_PLACEMENT_3D('',#248136,#136273,#136274);
#109102=AXIS2_PLACEMENT_3D('',#248137,#136275,#136276);
#109103=AXIS2_PLACEMENT_3D('',#248138,#136277,#136278);
#109104=AXIS2_PLACEMENT_3D('',#248139,#136279,#136280);
#109105=AXIS2_PLACEMENT_3D('',#248158,#136281,#136282);
#109106=AXIS2_PLACEMENT_3D('',#248159,#136283,#136284);
#109107=AXIS2_PLACEMENT_3D('',#248160,#136285,#136286);
#109108=AXIS2_PLACEMENT_3D('',#248161,#136287,#136288);
#109109=AXIS2_PLACEMENT_3D('',#248162,#136289,#136290);
#109110=AXIS2_PLACEMENT_3D('',#248175,#136291,#136292);
#109111=AXIS2_PLACEMENT_3D('',#248194,#136293,#136294);
#109112=AXIS2_PLACEMENT_3D('',#248195,#136295,#136296);
#109113=AXIS2_PLACEMENT_3D('',#248196,#136297,#136298);
#109114=AXIS2_PLACEMENT_3D('',#248197,#136299,#136300);
#109115=AXIS2_PLACEMENT_3D('',#248198,#136301,#136302);
#109116=AXIS2_PLACEMENT_3D('',#248217,#136303,#136304);
#109117=AXIS2_PLACEMENT_3D('',#248230,#136305,#136306);
#109118=AXIS2_PLACEMENT_3D('',#248231,#136307,#136308);
#109119=AXIS2_PLACEMENT_3D('',#248232,#136309,#136310);
#109120=AXIS2_PLACEMENT_3D('',#248233,#136311,#136312);
#109121=AXIS2_PLACEMENT_3D('',#248234,#136313,#136314);
#109122=AXIS2_PLACEMENT_3D('',#248253,#136315,#136316);
#109123=AXIS2_PLACEMENT_3D('',#248254,#136317,#136318);
#109124=AXIS2_PLACEMENT_3D('',#248255,#136319,#136320);
#109125=AXIS2_PLACEMENT_3D('',#248256,#136321,#136322);
#109126=AXIS2_PLACEMENT_3D('',#248257,#136323,#136324);
#109127=AXIS2_PLACEMENT_3D('',#248270,#136325,#136326);
#109128=AXIS2_PLACEMENT_3D('',#248283,#136327,#136328);
#109129=AXIS2_PLACEMENT_3D('',#248284,#136329,#136330);
#109130=AXIS2_PLACEMENT_3D('',#248285,#136331,#136332);
#109131=AXIS2_PLACEMENT_3D('',#248286,#136333,#136334);
#109132=AXIS2_PLACEMENT_3D('',#248287,#136335,#136336);
#109133=AXIS2_PLACEMENT_3D('',#248300,#136337,#136338);
#109134=AXIS2_PLACEMENT_3D('',#248301,#136339,#136340);
#109135=AXIS2_PLACEMENT_3D('',#248302,#136341,#136342);
#109136=AXIS2_PLACEMENT_3D('',#248303,#136343,#136344);
#109137=AXIS2_PLACEMENT_3D('',#248304,#136345,#136346);
#109138=AXIS2_PLACEMENT_3D('',#248317,#136347,#136348);
#109139=AXIS2_PLACEMENT_3D('',#248318,#136349,#136350);
#109140=AXIS2_PLACEMENT_3D('',#248319,#136351,#136352);
#109141=AXIS2_PLACEMENT_3D('',#248320,#136353,#136354);
#109142=AXIS2_PLACEMENT_3D('',#248321,#136355,#136356);
#109143=AXIS2_PLACEMENT_3D('',#248334,#136357,#136358);
#109144=AXIS2_PLACEMENT_3D('',#248347,#136359,#136360);
#109145=AXIS2_PLACEMENT_3D('',#248348,#136361,#136362);
#109146=AXIS2_PLACEMENT_3D('',#248349,#136363,#136364);
#109147=AXIS2_PLACEMENT_3D('',#248350,#136365,#136366);
#109148=AXIS2_PLACEMENT_3D('',#248351,#136367,#136368);
#109149=AXIS2_PLACEMENT_3D('',#248370,#136369,#136370);
#109150=AXIS2_PLACEMENT_3D('',#248371,#136371,#136372);
#109151=AXIS2_PLACEMENT_3D('',#248372,#136373,#136374);
#109152=AXIS2_PLACEMENT_3D('',#248373,#136375,#136376);
#109153=AXIS2_PLACEMENT_3D('',#248374,#136377,#136378);
#109154=AXIS2_PLACEMENT_3D('',#248387,#136379,#136380);
#109155=AXIS2_PLACEMENT_3D('',#248406,#136381,#136382);
#109156=AXIS2_PLACEMENT_3D('',#248407,#136383,#136384);
#109157=AXIS2_PLACEMENT_3D('',#248408,#136385,#136386);
#109158=AXIS2_PLACEMENT_3D('',#248409,#136387,#136388);
#109159=AXIS2_PLACEMENT_3D('',#248410,#136389,#136390);
#109160=AXIS2_PLACEMENT_3D('',#248429,#136391,#136392);
#109161=AXIS2_PLACEMENT_3D('',#248442,#136393,#136394);
#109162=AXIS2_PLACEMENT_3D('',#248443,#136395,#136396);
#109163=AXIS2_PLACEMENT_3D('',#248444,#136397,#136398);
#109164=AXIS2_PLACEMENT_3D('',#248445,#136399,#136400);
#109165=AXIS2_PLACEMENT_3D('',#248446,#136401,#136402);
#109166=AXIS2_PLACEMENT_3D('',#248465,#136403,#136404);
#109167=AXIS2_PLACEMENT_3D('',#248466,#136405,#136406);
#109168=AXIS2_PLACEMENT_3D('',#248467,#136407,#136408);
#109169=AXIS2_PLACEMENT_3D('',#248468,#136409,#136410);
#109170=AXIS2_PLACEMENT_3D('',#248469,#136411,#136412);
#109171=AXIS2_PLACEMENT_3D('',#248482,#136413,#136414);
#109172=AXIS2_PLACEMENT_3D('',#248495,#136415,#136416);
#109173=AXIS2_PLACEMENT_3D('',#248496,#136417,#136418);
#109174=AXIS2_PLACEMENT_3D('',#248497,#136419,#136420);
#109175=AXIS2_PLACEMENT_3D('',#248498,#136421,#136422);
#109176=AXIS2_PLACEMENT_3D('',#248499,#136423,#136424);
#109177=AXIS2_PLACEMENT_3D('',#248512,#136425,#136426);
#109178=AXIS2_PLACEMENT_3D('',#248513,#136427,#136428);
#109179=AXIS2_PLACEMENT_3D('',#248514,#136429,#136430);
#109180=AXIS2_PLACEMENT_3D('',#248515,#136431,#136432);
#109181=AXIS2_PLACEMENT_3D('',#248516,#136433,#136434);
#109182=AXIS2_PLACEMENT_3D('',#248529,#136435,#136436);
#109183=AXIS2_PLACEMENT_3D('',#248530,#136437,#136438);
#109184=AXIS2_PLACEMENT_3D('',#248531,#136439,#136440);
#109185=AXIS2_PLACEMENT_3D('',#248532,#136441,#136442);
#109186=AXIS2_PLACEMENT_3D('',#248533,#136443,#136444);
#109187=AXIS2_PLACEMENT_3D('',#248546,#136445,#136446);
#109188=AXIS2_PLACEMENT_3D('',#248559,#136447,#136448);
#109189=AXIS2_PLACEMENT_3D('',#248560,#136449,#136450);
#109190=AXIS2_PLACEMENT_3D('',#248561,#136451,#136452);
#109191=AXIS2_PLACEMENT_3D('',#248562,#136453,#136454);
#109192=AXIS2_PLACEMENT_3D('',#248563,#136455,#136456);
#109193=AXIS2_PLACEMENT_3D('',#248582,#136457,#136458);
#109194=AXIS2_PLACEMENT_3D('',#248583,#136459,#136460);
#109195=AXIS2_PLACEMENT_3D('',#248584,#136461,#136462);
#109196=AXIS2_PLACEMENT_3D('',#248585,#136463,#136464);
#109197=AXIS2_PLACEMENT_3D('',#248586,#136465,#136466);
#109198=AXIS2_PLACEMENT_3D('',#248599,#136467,#136468);
#109199=AXIS2_PLACEMENT_3D('',#248618,#136469,#136470);
#109200=AXIS2_PLACEMENT_3D('',#248619,#136471,#136472);
#109201=AXIS2_PLACEMENT_3D('',#248620,#136473,#136474);
#109202=AXIS2_PLACEMENT_3D('',#248621,#136475,#136476);
#109203=AXIS2_PLACEMENT_3D('',#248622,#136477,#136478);
#109204=AXIS2_PLACEMENT_3D('',#248641,#136479,#136480);
#109205=AXIS2_PLACEMENT_3D('',#248654,#136481,#136482);
#109206=AXIS2_PLACEMENT_3D('',#248655,#136483,#136484);
#109207=AXIS2_PLACEMENT_3D('',#248656,#136485,#136486);
#109208=AXIS2_PLACEMENT_3D('',#248657,#136487,#136488);
#109209=AXIS2_PLACEMENT_3D('',#248658,#136489,#136490);
#109210=AXIS2_PLACEMENT_3D('',#248677,#136491,#136492);
#109211=AXIS2_PLACEMENT_3D('',#248678,#136493,#136494);
#109212=AXIS2_PLACEMENT_3D('',#248679,#136495,#136496);
#109213=AXIS2_PLACEMENT_3D('',#248680,#136497,#136498);
#109214=AXIS2_PLACEMENT_3D('',#248681,#136499,#136500);
#109215=AXIS2_PLACEMENT_3D('',#248694,#136501,#136502);
#109216=AXIS2_PLACEMENT_3D('',#248707,#136503,#136504);
#109217=AXIS2_PLACEMENT_3D('',#248708,#136505,#136506);
#109218=AXIS2_PLACEMENT_3D('',#248709,#136507,#136508);
#109219=AXIS2_PLACEMENT_3D('',#248710,#136509,#136510);
#109220=AXIS2_PLACEMENT_3D('',#248711,#136511,#136512);
#109221=AXIS2_PLACEMENT_3D('',#248724,#136513,#136514);
#109222=AXIS2_PLACEMENT_3D('',#248725,#136515,#136516);
#109223=AXIS2_PLACEMENT_3D('',#248726,#136517,#136518);
#109224=AXIS2_PLACEMENT_3D('',#248727,#136519,#136520);
#109225=AXIS2_PLACEMENT_3D('',#248728,#136521,#136522);
#109226=AXIS2_PLACEMENT_3D('',#248741,#136523,#136524);
#109227=AXIS2_PLACEMENT_3D('',#248742,#136525,#136526);
#109228=AXIS2_PLACEMENT_3D('',#248743,#136527,#136528);
#109229=AXIS2_PLACEMENT_3D('',#248744,#136529,#136530);
#109230=AXIS2_PLACEMENT_3D('',#248745,#136531,#136532);
#109231=AXIS2_PLACEMENT_3D('',#248758,#136533,#136534);
#109232=AXIS2_PLACEMENT_3D('',#248771,#136535,#136536);
#109233=AXIS2_PLACEMENT_3D('',#248772,#136537,#136538);
#109234=AXIS2_PLACEMENT_3D('',#248773,#136539,#136540);
#109235=AXIS2_PLACEMENT_3D('',#248774,#136541,#136542);
#109236=AXIS2_PLACEMENT_3D('',#248775,#136543,#136544);
#109237=AXIS2_PLACEMENT_3D('',#248794,#136545,#136546);
#109238=AXIS2_PLACEMENT_3D('',#248795,#136547,#136548);
#109239=AXIS2_PLACEMENT_3D('',#248796,#136549,#136550);
#109240=AXIS2_PLACEMENT_3D('',#248797,#136551,#136552);
#109241=AXIS2_PLACEMENT_3D('',#248798,#136553,#136554);
#109242=AXIS2_PLACEMENT_3D('',#248811,#136555,#136556);
#109243=AXIS2_PLACEMENT_3D('',#248830,#136557,#136558);
#109244=AXIS2_PLACEMENT_3D('',#248831,#136559,#136560);
#109245=AXIS2_PLACEMENT_3D('',#248832,#136561,#136562);
#109246=AXIS2_PLACEMENT_3D('',#248833,#136563,#136564);
#109247=AXIS2_PLACEMENT_3D('',#248834,#136565,#136566);
#109248=AXIS2_PLACEMENT_3D('',#248853,#136567,#136568);
#109249=AXIS2_PLACEMENT_3D('',#248866,#136569,#136570);
#109250=AXIS2_PLACEMENT_3D('',#248867,#136571,#136572);
#109251=AXIS2_PLACEMENT_3D('',#248868,#136573,#136574);
#109252=AXIS2_PLACEMENT_3D('',#248869,#136575,#136576);
#109253=AXIS2_PLACEMENT_3D('',#248870,#136577,#136578);
#109254=AXIS2_PLACEMENT_3D('',#248889,#136579,#136580);
#109255=AXIS2_PLACEMENT_3D('',#248890,#136581,#136582);
#109256=AXIS2_PLACEMENT_3D('',#248891,#136583,#136584);
#109257=AXIS2_PLACEMENT_3D('',#248892,#136585,#136586);
#109258=AXIS2_PLACEMENT_3D('',#248893,#136587,#136588);
#109259=AXIS2_PLACEMENT_3D('',#248906,#136589,#136590);
#109260=AXIS2_PLACEMENT_3D('',#248919,#136591,#136592);
#109261=AXIS2_PLACEMENT_3D('',#248920,#136593,#136594);
#109262=AXIS2_PLACEMENT_3D('',#248921,#136595,#136596);
#109263=AXIS2_PLACEMENT_3D('',#248922,#136597,#136598);
#109264=AXIS2_PLACEMENT_3D('',#248923,#136599,#136600);
#109265=AXIS2_PLACEMENT_3D('',#248936,#136601,#136602);
#109266=AXIS2_PLACEMENT_3D('',#248937,#136603,#136604);
#109267=AXIS2_PLACEMENT_3D('',#248938,#136605,#136606);
#109268=AXIS2_PLACEMENT_3D('',#248939,#136607,#136608);
#109269=AXIS2_PLACEMENT_3D('',#248940,#136609,#136610);
#109270=AXIS2_PLACEMENT_3D('',#248953,#136611,#136612);
#109271=AXIS2_PLACEMENT_3D('',#248954,#136613,#136614);
#109272=AXIS2_PLACEMENT_3D('',#248955,#136615,#136616);
#109273=AXIS2_PLACEMENT_3D('',#248956,#136617,#136618);
#109274=AXIS2_PLACEMENT_3D('',#248957,#136619,#136620);
#109275=AXIS2_PLACEMENT_3D('',#248970,#136621,#136622);
#109276=AXIS2_PLACEMENT_3D('',#248983,#136623,#136624);
#109277=AXIS2_PLACEMENT_3D('',#248984,#136625,#136626);
#109278=AXIS2_PLACEMENT_3D('',#248985,#136627,#136628);
#109279=AXIS2_PLACEMENT_3D('',#248986,#136629,#136630);
#109280=AXIS2_PLACEMENT_3D('',#248987,#136631,#136632);
#109281=AXIS2_PLACEMENT_3D('',#249006,#136633,#136634);
#109282=AXIS2_PLACEMENT_3D('',#249007,#136635,#136636);
#109283=AXIS2_PLACEMENT_3D('',#249008,#136637,#136638);
#109284=AXIS2_PLACEMENT_3D('',#249009,#136639,#136640);
#109285=AXIS2_PLACEMENT_3D('',#249010,#136641,#136642);
#109286=AXIS2_PLACEMENT_3D('',#249023,#136643,#136644);
#109287=AXIS2_PLACEMENT_3D('',#249042,#136645,#136646);
#109288=AXIS2_PLACEMENT_3D('',#249043,#136647,#136648);
#109289=AXIS2_PLACEMENT_3D('',#249044,#136649,#136650);
#109290=AXIS2_PLACEMENT_3D('',#249045,#136651,#136652);
#109291=AXIS2_PLACEMENT_3D('',#249046,#136653,#136654);
#109292=AXIS2_PLACEMENT_3D('',#249065,#136655,#136656);
#109293=AXIS2_PLACEMENT_3D('',#249078,#136657,#136658);
#109294=AXIS2_PLACEMENT_3D('',#249079,#136659,#136660);
#109295=AXIS2_PLACEMENT_3D('',#249080,#136661,#136662);
#109296=AXIS2_PLACEMENT_3D('',#249081,#136663,#136664);
#109297=AXIS2_PLACEMENT_3D('',#249082,#136665,#136666);
#109298=AXIS2_PLACEMENT_3D('',#249101,#136667,#136668);
#109299=AXIS2_PLACEMENT_3D('',#249102,#136669,#136670);
#109300=AXIS2_PLACEMENT_3D('',#249103,#136671,#136672);
#109301=AXIS2_PLACEMENT_3D('',#249104,#136673,#136674);
#109302=AXIS2_PLACEMENT_3D('',#249105,#136675,#136676);
#109303=AXIS2_PLACEMENT_3D('',#249118,#136677,#136678);
#109304=AXIS2_PLACEMENT_3D('',#249131,#136679,#136680);
#109305=AXIS2_PLACEMENT_3D('',#249132,#136681,#136682);
#109306=AXIS2_PLACEMENT_3D('',#249133,#136683,#136684);
#109307=AXIS2_PLACEMENT_3D('',#249134,#136685,#136686);
#109308=AXIS2_PLACEMENT_3D('',#249135,#136687,#136688);
#109309=AXIS2_PLACEMENT_3D('',#249148,#136689,#136690);
#109310=AXIS2_PLACEMENT_3D('',#249149,#136691,#136692);
#109311=AXIS2_PLACEMENT_3D('',#249150,#136693,#136694);
#109312=AXIS2_PLACEMENT_3D('',#249151,#136695,#136696);
#109313=AXIS2_PLACEMENT_3D('',#249152,#136697,#136698);
#109314=AXIS2_PLACEMENT_3D('',#249165,#136699,#136700);
#109315=AXIS2_PLACEMENT_3D('',#249166,#136701,#136702);
#109316=AXIS2_PLACEMENT_3D('',#249167,#136703,#136704);
#109317=AXIS2_PLACEMENT_3D('',#249168,#136705,#136706);
#109318=AXIS2_PLACEMENT_3D('',#249169,#136707,#136708);
#109319=AXIS2_PLACEMENT_3D('',#249182,#136709,#136710);
#109320=AXIS2_PLACEMENT_3D('',#249195,#136711,#136712);
#109321=AXIS2_PLACEMENT_3D('',#249196,#136713,#136714);
#109322=AXIS2_PLACEMENT_3D('',#249197,#136715,#136716);
#109323=AXIS2_PLACEMENT_3D('',#249198,#136717,#136718);
#109324=AXIS2_PLACEMENT_3D('',#249199,#136719,#136720);
#109325=AXIS2_PLACEMENT_3D('',#249218,#136721,#136722);
#109326=AXIS2_PLACEMENT_3D('',#249219,#136723,#136724);
#109327=AXIS2_PLACEMENT_3D('',#249220,#136725,#136726);
#109328=AXIS2_PLACEMENT_3D('',#249221,#136727,#136728);
#109329=AXIS2_PLACEMENT_3D('',#249222,#136729,#136730);
#109330=AXIS2_PLACEMENT_3D('',#249235,#136731,#136732);
#109331=AXIS2_PLACEMENT_3D('',#249254,#136733,#136734);
#109332=AXIS2_PLACEMENT_3D('',#249255,#136735,#136736);
#109333=AXIS2_PLACEMENT_3D('',#249256,#136737,#136738);
#109334=AXIS2_PLACEMENT_3D('',#249257,#136739,#136740);
#109335=AXIS2_PLACEMENT_3D('',#249258,#136741,#136742);
#109336=AXIS2_PLACEMENT_3D('',#249277,#136743,#136744);
#109337=AXIS2_PLACEMENT_3D('',#249290,#136745,#136746);
#109338=AXIS2_PLACEMENT_3D('',#249291,#136747,#136748);
#109339=AXIS2_PLACEMENT_3D('',#249292,#136749,#136750);
#109340=AXIS2_PLACEMENT_3D('',#249293,#136751,#136752);
#109341=AXIS2_PLACEMENT_3D('',#249294,#136753,#136754);
#109342=AXIS2_PLACEMENT_3D('',#249313,#136755,#136756);
#109343=AXIS2_PLACEMENT_3D('',#249314,#136757,#136758);
#109344=AXIS2_PLACEMENT_3D('',#249315,#136759,#136760);
#109345=AXIS2_PLACEMENT_3D('',#249316,#136761,#136762);
#109346=AXIS2_PLACEMENT_3D('',#249317,#136763,#136764);
#109347=AXIS2_PLACEMENT_3D('',#249330,#136765,#136766);
#109348=AXIS2_PLACEMENT_3D('',#249343,#136767,#136768);
#109349=AXIS2_PLACEMENT_3D('',#249344,#136769,#136770);
#109350=AXIS2_PLACEMENT_3D('',#249345,#136771,#136772);
#109351=AXIS2_PLACEMENT_3D('',#249346,#136773,#136774);
#109352=AXIS2_PLACEMENT_3D('',#249347,#136775,#136776);
#109353=AXIS2_PLACEMENT_3D('',#249360,#136777,#136778);
#109354=AXIS2_PLACEMENT_3D('',#249361,#136779,#136780);
#109355=AXIS2_PLACEMENT_3D('',#249362,#136781,#136782);
#109356=AXIS2_PLACEMENT_3D('',#249363,#136783,#136784);
#109357=AXIS2_PLACEMENT_3D('',#249364,#136785,#136786);
#109358=AXIS2_PLACEMENT_3D('',#249377,#136787,#136788);
#109359=AXIS2_PLACEMENT_3D('',#249378,#136789,#136790);
#109360=AXIS2_PLACEMENT_3D('',#249379,#136791,#136792);
#109361=AXIS2_PLACEMENT_3D('',#249380,#136793,#136794);
#109362=AXIS2_PLACEMENT_3D('',#249381,#136795,#136796);
#109363=AXIS2_PLACEMENT_3D('',#249394,#136797,#136798);
#109364=AXIS2_PLACEMENT_3D('',#249407,#136799,#136800);
#109365=AXIS2_PLACEMENT_3D('',#249408,#136801,#136802);
#109366=AXIS2_PLACEMENT_3D('',#249409,#136803,#136804);
#109367=AXIS2_PLACEMENT_3D('',#249410,#136805,#136806);
#109368=AXIS2_PLACEMENT_3D('',#249411,#136807,#136808);
#109369=AXIS2_PLACEMENT_3D('',#249430,#136809,#136810);
#109370=AXIS2_PLACEMENT_3D('',#249431,#136811,#136812);
#109371=AXIS2_PLACEMENT_3D('',#249432,#136813,#136814);
#109372=AXIS2_PLACEMENT_3D('',#249433,#136815,#136816);
#109373=AXIS2_PLACEMENT_3D('',#249434,#136817,#136818);
#109374=AXIS2_PLACEMENT_3D('',#249447,#136819,#136820);
#109375=AXIS2_PLACEMENT_3D('',#249466,#136821,#136822);
#109376=AXIS2_PLACEMENT_3D('',#249467,#136823,#136824);
#109377=AXIS2_PLACEMENT_3D('',#249468,#136825,#136826);
#109378=AXIS2_PLACEMENT_3D('',#249469,#136827,#136828);
#109379=AXIS2_PLACEMENT_3D('',#249470,#136829,#136830);
#109380=AXIS2_PLACEMENT_3D('',#249489,#136831,#136832);
#109381=AXIS2_PLACEMENT_3D('',#249502,#136833,#136834);
#109382=AXIS2_PLACEMENT_3D('',#249503,#136835,#136836);
#109383=AXIS2_PLACEMENT_3D('',#249504,#136837,#136838);
#109384=AXIS2_PLACEMENT_3D('',#249505,#136839,#136840);
#109385=AXIS2_PLACEMENT_3D('',#249506,#136841,#136842);
#109386=AXIS2_PLACEMENT_3D('',#249525,#136843,#136844);
#109387=AXIS2_PLACEMENT_3D('',#249526,#136845,#136846);
#109388=AXIS2_PLACEMENT_3D('',#249527,#136847,#136848);
#109389=AXIS2_PLACEMENT_3D('',#249528,#136849,#136850);
#109390=AXIS2_PLACEMENT_3D('',#249529,#136851,#136852);
#109391=AXIS2_PLACEMENT_3D('',#249542,#136853,#136854);
#109392=AXIS2_PLACEMENT_3D('',#249555,#136855,#136856);
#109393=AXIS2_PLACEMENT_3D('',#249556,#136857,#136858);
#109394=AXIS2_PLACEMENT_3D('',#249557,#136859,#136860);
#109395=AXIS2_PLACEMENT_3D('',#249558,#136861,#136862);
#109396=AXIS2_PLACEMENT_3D('',#249559,#136863,#136864);
#109397=AXIS2_PLACEMENT_3D('',#249572,#136865,#136866);
#109398=AXIS2_PLACEMENT_3D('',#249573,#136867,#136868);
#109399=AXIS2_PLACEMENT_3D('',#249574,#136869,#136870);
#109400=AXIS2_PLACEMENT_3D('',#249575,#136871,#136872);
#109401=AXIS2_PLACEMENT_3D('',#249576,#136873,#136874);
#109402=AXIS2_PLACEMENT_3D('',#249589,#136875,#136876);
#109403=AXIS2_PLACEMENT_3D('',#249590,#136877,#136878);
#109404=AXIS2_PLACEMENT_3D('',#249591,#136879,#136880);
#109405=AXIS2_PLACEMENT_3D('',#249592,#136881,#136882);
#109406=AXIS2_PLACEMENT_3D('',#249593,#136883,#136884);
#109407=AXIS2_PLACEMENT_3D('',#249606,#136885,#136886);
#109408=AXIS2_PLACEMENT_3D('',#249619,#136887,#136888);
#109409=AXIS2_PLACEMENT_3D('',#249620,#136889,#136890);
#109410=AXIS2_PLACEMENT_3D('',#249621,#136891,#136892);
#109411=AXIS2_PLACEMENT_3D('',#249622,#136893,#136894);
#109412=AXIS2_PLACEMENT_3D('',#249623,#136895,#136896);
#109413=AXIS2_PLACEMENT_3D('',#249642,#136897,#136898);
#109414=AXIS2_PLACEMENT_3D('',#249643,#136899,#136900);
#109415=AXIS2_PLACEMENT_3D('',#249644,#136901,#136902);
#109416=AXIS2_PLACEMENT_3D('',#249645,#136903,#136904);
#109417=AXIS2_PLACEMENT_3D('',#249646,#136905,#136906);
#109418=AXIS2_PLACEMENT_3D('',#249659,#136907,#136908);
#109419=AXIS2_PLACEMENT_3D('',#249678,#136909,#136910);
#109420=AXIS2_PLACEMENT_3D('',#249679,#136911,#136912);
#109421=AXIS2_PLACEMENT_3D('',#249680,#136913,#136914);
#109422=AXIS2_PLACEMENT_3D('',#249681,#136915,#136916);
#109423=AXIS2_PLACEMENT_3D('',#249682,#136917,#136918);
#109424=AXIS2_PLACEMENT_3D('',#249701,#136919,#136920);
#109425=AXIS2_PLACEMENT_3D('',#249714,#136921,#136922);
#109426=AXIS2_PLACEMENT_3D('',#249715,#136923,#136924);
#109427=AXIS2_PLACEMENT_3D('',#249716,#136925,#136926);
#109428=AXIS2_PLACEMENT_3D('',#249717,#136927,#136928);
#109429=AXIS2_PLACEMENT_3D('',#249718,#136929,#136930);
#109430=AXIS2_PLACEMENT_3D('',#249737,#136931,#136932);
#109431=AXIS2_PLACEMENT_3D('',#249738,#136933,#136934);
#109432=AXIS2_PLACEMENT_3D('',#249739,#136935,#136936);
#109433=AXIS2_PLACEMENT_3D('',#249740,#136937,#136938);
#109434=AXIS2_PLACEMENT_3D('',#249741,#136939,#136940);
#109435=AXIS2_PLACEMENT_3D('',#249754,#136941,#136942);
#109436=AXIS2_PLACEMENT_3D('',#249767,#136943,#136944);
#109437=AXIS2_PLACEMENT_3D('',#249768,#136945,#136946);
#109438=AXIS2_PLACEMENT_3D('',#249769,#136947,#136948);
#109439=AXIS2_PLACEMENT_3D('',#249770,#136949,#136950);
#109440=AXIS2_PLACEMENT_3D('',#249771,#136951,#136952);
#109441=AXIS2_PLACEMENT_3D('',#249784,#136953,#136954);
#109442=AXIS2_PLACEMENT_3D('',#249785,#136955,#136956);
#109443=AXIS2_PLACEMENT_3D('',#249786,#136957,#136958);
#109444=AXIS2_PLACEMENT_3D('',#249787,#136959,#136960);
#109445=AXIS2_PLACEMENT_3D('',#249788,#136961,#136962);
#109446=AXIS2_PLACEMENT_3D('',#249801,#136963,#136964);
#109447=AXIS2_PLACEMENT_3D('',#249802,#136965,#136966);
#109448=AXIS2_PLACEMENT_3D('',#249803,#136967,#136968);
#109449=AXIS2_PLACEMENT_3D('',#249804,#136969,#136970);
#109450=AXIS2_PLACEMENT_3D('',#249805,#136971,#136972);
#109451=AXIS2_PLACEMENT_3D('',#249818,#136973,#136974);
#109452=AXIS2_PLACEMENT_3D('',#249831,#136975,#136976);
#109453=AXIS2_PLACEMENT_3D('',#249832,#136977,#136978);
#109454=AXIS2_PLACEMENT_3D('',#249833,#136979,#136980);
#109455=AXIS2_PLACEMENT_3D('',#249834,#136981,#136982);
#109456=AXIS2_PLACEMENT_3D('',#249835,#136983,#136984);
#109457=AXIS2_PLACEMENT_3D('',#249854,#136985,#136986);
#109458=AXIS2_PLACEMENT_3D('',#249855,#136987,#136988);
#109459=AXIS2_PLACEMENT_3D('',#249856,#136989,#136990);
#109460=AXIS2_PLACEMENT_3D('',#249857,#136991,#136992);
#109461=AXIS2_PLACEMENT_3D('',#249858,#136993,#136994);
#109462=AXIS2_PLACEMENT_3D('',#249871,#136995,#136996);
#109463=AXIS2_PLACEMENT_3D('',#249890,#136997,#136998);
#109464=AXIS2_PLACEMENT_3D('',#249891,#136999,#137000);
#109465=AXIS2_PLACEMENT_3D('',#249892,#137001,#137002);
#109466=AXIS2_PLACEMENT_3D('',#249893,#137003,#137004);
#109467=AXIS2_PLACEMENT_3D('',#249894,#137005,#137006);
#109468=AXIS2_PLACEMENT_3D('',#249913,#137007,#137008);
#109469=AXIS2_PLACEMENT_3D('',#249926,#137009,#137010);
#109470=AXIS2_PLACEMENT_3D('',#249927,#137011,#137012);
#109471=AXIS2_PLACEMENT_3D('',#249928,#137013,#137014);
#109472=AXIS2_PLACEMENT_3D('',#249929,#137015,#137016);
#109473=AXIS2_PLACEMENT_3D('',#249930,#137017,#137018);
#109474=AXIS2_PLACEMENT_3D('',#249949,#137019,#137020);
#109475=AXIS2_PLACEMENT_3D('',#249950,#137021,#137022);
#109476=AXIS2_PLACEMENT_3D('',#249951,#137023,#137024);
#109477=AXIS2_PLACEMENT_3D('',#249952,#137025,#137026);
#109478=AXIS2_PLACEMENT_3D('',#249953,#137027,#137028);
#109479=AXIS2_PLACEMENT_3D('',#249966,#137029,#137030);
#109480=AXIS2_PLACEMENT_3D('',#249979,#137031,#137032);
#109481=AXIS2_PLACEMENT_3D('',#249980,#137033,#137034);
#109482=AXIS2_PLACEMENT_3D('',#249981,#137035,#137036);
#109483=AXIS2_PLACEMENT_3D('',#249982,#137037,#137038);
#109484=AXIS2_PLACEMENT_3D('',#249983,#137039,#137040);
#109485=AXIS2_PLACEMENT_3D('',#249996,#137041,#137042);
#109486=AXIS2_PLACEMENT_3D('',#249997,#137043,#137044);
#109487=AXIS2_PLACEMENT_3D('',#249998,#137045,#137046);
#109488=AXIS2_PLACEMENT_3D('',#249999,#137047,#137048);
#109489=AXIS2_PLACEMENT_3D('',#250000,#137049,#137050);
#109490=AXIS2_PLACEMENT_3D('',#250013,#137051,#137052);
#109491=AXIS2_PLACEMENT_3D('',#250014,#137053,#137054);
#109492=AXIS2_PLACEMENT_3D('',#250015,#137055,#137056);
#109493=AXIS2_PLACEMENT_3D('',#250016,#137057,#137058);
#109494=AXIS2_PLACEMENT_3D('',#250017,#137059,#137060);
#109495=AXIS2_PLACEMENT_3D('',#250030,#137061,#137062);
#109496=AXIS2_PLACEMENT_3D('',#250043,#137063,#137064);
#109497=AXIS2_PLACEMENT_3D('',#250044,#137065,#137066);
#109498=AXIS2_PLACEMENT_3D('',#250045,#137067,#137068);
#109499=AXIS2_PLACEMENT_3D('',#250046,#137069,#137070);
#109500=AXIS2_PLACEMENT_3D('',#250047,#137071,#137072);
#109501=AXIS2_PLACEMENT_3D('',#250066,#137073,#137074);
#109502=AXIS2_PLACEMENT_3D('',#250067,#137075,#137076);
#109503=AXIS2_PLACEMENT_3D('',#250068,#137077,#137078);
#109504=AXIS2_PLACEMENT_3D('',#250069,#137079,#137080);
#109505=AXIS2_PLACEMENT_3D('',#250070,#137081,#137082);
#109506=AXIS2_PLACEMENT_3D('',#250083,#137083,#137084);
#109507=AXIS2_PLACEMENT_3D('',#250102,#137085,#137086);
#109508=AXIS2_PLACEMENT_3D('',#250103,#137087,#137088);
#109509=AXIS2_PLACEMENT_3D('',#250104,#137089,#137090);
#109510=AXIS2_PLACEMENT_3D('',#250105,#137091,#137092);
#109511=AXIS2_PLACEMENT_3D('',#250106,#137093,#137094);
#109512=AXIS2_PLACEMENT_3D('',#250125,#137095,#137096);
#109513=AXIS2_PLACEMENT_3D('',#250138,#137097,#137098);
#109514=AXIS2_PLACEMENT_3D('',#250139,#137099,#137100);
#109515=AXIS2_PLACEMENT_3D('',#250140,#137101,#137102);
#109516=AXIS2_PLACEMENT_3D('',#250141,#137103,#137104);
#109517=AXIS2_PLACEMENT_3D('',#250142,#137105,#137106);
#109518=AXIS2_PLACEMENT_3D('',#250161,#137107,#137108);
#109519=AXIS2_PLACEMENT_3D('',#250162,#137109,#137110);
#109520=AXIS2_PLACEMENT_3D('',#250163,#137111,#137112);
#109521=AXIS2_PLACEMENT_3D('',#250164,#137113,#137114);
#109522=AXIS2_PLACEMENT_3D('',#250165,#137115,#137116);
#109523=AXIS2_PLACEMENT_3D('',#250178,#137117,#137118);
#109524=AXIS2_PLACEMENT_3D('',#250191,#137119,#137120);
#109525=AXIS2_PLACEMENT_3D('',#250192,#137121,#137122);
#109526=AXIS2_PLACEMENT_3D('',#250193,#137123,#137124);
#109527=AXIS2_PLACEMENT_3D('',#250194,#137125,#137126);
#109528=AXIS2_PLACEMENT_3D('',#250195,#137127,#137128);
#109529=AXIS2_PLACEMENT_3D('',#250208,#137129,#137130);
#109530=AXIS2_PLACEMENT_3D('',#250209,#137131,#137132);
#109531=AXIS2_PLACEMENT_3D('',#250210,#137133,#137134);
#109532=AXIS2_PLACEMENT_3D('',#250211,#137135,#137136);
#109533=AXIS2_PLACEMENT_3D('',#250212,#137137,#137138);
#109534=AXIS2_PLACEMENT_3D('',#250225,#137139,#137140);
#109535=AXIS2_PLACEMENT_3D('',#250226,#137141,#137142);
#109536=AXIS2_PLACEMENT_3D('',#250227,#137143,#137144);
#109537=AXIS2_PLACEMENT_3D('',#250228,#137145,#137146);
#109538=AXIS2_PLACEMENT_3D('',#250229,#137147,#137148);
#109539=AXIS2_PLACEMENT_3D('',#250242,#137149,#137150);
#109540=AXIS2_PLACEMENT_3D('',#250255,#137151,#137152);
#109541=AXIS2_PLACEMENT_3D('',#250256,#137153,#137154);
#109542=AXIS2_PLACEMENT_3D('',#250257,#137155,#137156);
#109543=AXIS2_PLACEMENT_3D('',#250258,#137157,#137158);
#109544=AXIS2_PLACEMENT_3D('',#250259,#137159,#137160);
#109545=AXIS2_PLACEMENT_3D('',#250278,#137161,#137162);
#109546=AXIS2_PLACEMENT_3D('',#250279,#137163,#137164);
#109547=AXIS2_PLACEMENT_3D('',#250292,#137165,#137166);
#109548=AXIS2_PLACEMENT_3D('',#250311,#137167,#137168);
#109549=AXIS2_PLACEMENT_3D('',#250312,#137169,#137170);
#109550=AXIS2_PLACEMENT_3D('',#250313,#137171,#137172);
#109551=AXIS2_PLACEMENT_3D('',#250314,#137173,#137174);
#109552=AXIS2_PLACEMENT_3D('',#250315,#137175,#137176);
#109553=AXIS2_PLACEMENT_3D('',#250346,#137177,#137178);
#109554=AXIS2_PLACEMENT_3D('',#250347,#137179,#137180);
#109555=AXIS2_PLACEMENT_3D('',#250348,#137181,#137182);
#109556=AXIS2_PLACEMENT_3D('',#250367,#137183,#137184);
#109557=AXIS2_PLACEMENT_3D('',#250368,#137185,#137186);
#109558=AXIS2_PLACEMENT_3D('',#250369,#137187,#137188);
#109559=AXIS2_PLACEMENT_3D('',#250370,#137189,#137190);
#109560=AXIS2_PLACEMENT_3D('',#250371,#137191,#137192);
#109561=AXIS2_PLACEMENT_3D('',#250384,#137193,#137194);
#109562=AXIS2_PLACEMENT_3D('',#250397,#137195,#137196);
#109563=AXIS2_PLACEMENT_3D('',#250398,#137197,#137198);
#109564=AXIS2_PLACEMENT_3D('',#250399,#137199,#137200);
#109565=AXIS2_PLACEMENT_3D('',#250400,#137201,#137202);
#109566=AXIS2_PLACEMENT_3D('',#250401,#137203,#137204);
#109567=AXIS2_PLACEMENT_3D('',#250414,#137205,#137206);
#109568=AXIS2_PLACEMENT_3D('',#250415,#137207,#137208);
#109569=AXIS2_PLACEMENT_3D('',#250416,#137209,#137210);
#109570=AXIS2_PLACEMENT_3D('',#250417,#137211,#137212);
#109571=AXIS2_PLACEMENT_3D('',#250418,#137213,#137214);
#109572=AXIS2_PLACEMENT_3D('',#250431,#137215,#137216);
#109573=AXIS2_PLACEMENT_3D('',#250432,#137217,#137218);
#109574=AXIS2_PLACEMENT_3D('',#250433,#137219,#137220);
#109575=AXIS2_PLACEMENT_3D('',#250434,#137221,#137222);
#109576=AXIS2_PLACEMENT_3D('',#250435,#137223,#137224);
#109577=AXIS2_PLACEMENT_3D('',#250448,#137225,#137226);
#109578=AXIS2_PLACEMENT_3D('',#250461,#137227,#137228);
#109579=AXIS2_PLACEMENT_3D('',#250462,#137229,#137230);
#109580=AXIS2_PLACEMENT_3D('',#250463,#137231,#137232);
#109581=AXIS2_PLACEMENT_3D('',#250464,#137233,#137234);
#109582=AXIS2_PLACEMENT_3D('',#250465,#137235,#137236);
#109583=AXIS2_PLACEMENT_3D('',#250484,#137237,#137238);
#109584=AXIS2_PLACEMENT_3D('',#250485,#137239,#137240);
#109585=AXIS2_PLACEMENT_3D('',#250486,#137241,#137242);
#109586=AXIS2_PLACEMENT_3D('',#250487,#137243,#137244);
#109587=AXIS2_PLACEMENT_3D('',#250488,#137245,#137246);
#109588=AXIS2_PLACEMENT_3D('',#250501,#137247,#137248);
#109589=AXIS2_PLACEMENT_3D('',#250520,#137249,#137250);
#109590=AXIS2_PLACEMENT_3D('',#250521,#137251,#137252);
#109591=AXIS2_PLACEMENT_3D('',#250522,#137253,#137254);
#109592=AXIS2_PLACEMENT_3D('',#250523,#137255,#137256);
#109593=AXIS2_PLACEMENT_3D('',#250524,#137257,#137258);
#109594=AXIS2_PLACEMENT_3D('',#250543,#137259,#137260);
#109595=AXIS2_PLACEMENT_3D('',#250556,#137261,#137262);
#109596=AXIS2_PLACEMENT_3D('',#250557,#137263,#137264);
#109597=AXIS2_PLACEMENT_3D('',#250558,#137265,#137266);
#109598=AXIS2_PLACEMENT_3D('',#250559,#137267,#137268);
#109599=AXIS2_PLACEMENT_3D('',#250560,#137269,#137270);
#109600=AXIS2_PLACEMENT_3D('',#250579,#137271,#137272);
#109601=AXIS2_PLACEMENT_3D('',#250580,#137273,#137274);
#109602=AXIS2_PLACEMENT_3D('',#250581,#137275,#137276);
#109603=AXIS2_PLACEMENT_3D('',#250582,#137277,#137278);
#109604=AXIS2_PLACEMENT_3D('',#250583,#137279,#137280);
#109605=AXIS2_PLACEMENT_3D('',#250596,#137281,#137282);
#109606=AXIS2_PLACEMENT_3D('',#250609,#137283,#137284);
#109607=AXIS2_PLACEMENT_3D('',#250610,#137285,#137286);
#109608=AXIS2_PLACEMENT_3D('',#250611,#137287,#137288);
#109609=AXIS2_PLACEMENT_3D('',#250612,#137289,#137290);
#109610=AXIS2_PLACEMENT_3D('',#250613,#137291,#137292);
#109611=AXIS2_PLACEMENT_3D('',#250626,#137293,#137294);
#109612=AXIS2_PLACEMENT_3D('',#250627,#137295,#137296);
#109613=AXIS2_PLACEMENT_3D('',#250628,#137297,#137298);
#109614=AXIS2_PLACEMENT_3D('',#250629,#137299,#137300);
#109615=AXIS2_PLACEMENT_3D('',#250630,#137301,#137302);
#109616=AXIS2_PLACEMENT_3D('',#250643,#137303,#137304);
#109617=AXIS2_PLACEMENT_3D('',#250644,#137305,#137306);
#109618=AXIS2_PLACEMENT_3D('',#250645,#137307,#137308);
#109619=AXIS2_PLACEMENT_3D('',#250646,#137309,#137310);
#109620=AXIS2_PLACEMENT_3D('',#250647,#137311,#137312);
#109621=AXIS2_PLACEMENT_3D('',#250660,#137313,#137314);
#109622=AXIS2_PLACEMENT_3D('',#250673,#137315,#137316);
#109623=AXIS2_PLACEMENT_3D('',#250674,#137317,#137318);
#109624=AXIS2_PLACEMENT_3D('',#250675,#137319,#137320);
#109625=AXIS2_PLACEMENT_3D('',#250676,#137321,#137322);
#109626=AXIS2_PLACEMENT_3D('',#250677,#137323,#137324);
#109627=AXIS2_PLACEMENT_3D('',#250696,#137325,#137326);
#109628=AXIS2_PLACEMENT_3D('',#250697,#137327,#137328);
#109629=AXIS2_PLACEMENT_3D('',#250698,#137329,#137330);
#109630=AXIS2_PLACEMENT_3D('',#250699,#137331,#137332);
#109631=AXIS2_PLACEMENT_3D('',#250700,#137333,#137334);
#109632=AXIS2_PLACEMENT_3D('',#250713,#137335,#137336);
#109633=AXIS2_PLACEMENT_3D('',#250732,#137337,#137338);
#109634=AXIS2_PLACEMENT_3D('',#250733,#137339,#137340);
#109635=AXIS2_PLACEMENT_3D('',#250734,#137341,#137342);
#109636=AXIS2_PLACEMENT_3D('',#250735,#137343,#137344);
#109637=AXIS2_PLACEMENT_3D('',#250736,#137345,#137346);
#109638=AXIS2_PLACEMENT_3D('',#250755,#137347,#137348);
#109639=AXIS2_PLACEMENT_3D('',#250768,#137349,#137350);
#109640=AXIS2_PLACEMENT_3D('',#250769,#137351,#137352);
#109641=AXIS2_PLACEMENT_3D('',#250770,#137353,#137354);
#109642=AXIS2_PLACEMENT_3D('',#250771,#137355,#137356);
#109643=AXIS2_PLACEMENT_3D('',#250772,#137357,#137358);
#109644=AXIS2_PLACEMENT_3D('',#250791,#137359,#137360);
#109645=AXIS2_PLACEMENT_3D('',#250792,#137361,#137362);
#109646=AXIS2_PLACEMENT_3D('',#250793,#137363,#137364);
#109647=AXIS2_PLACEMENT_3D('',#250794,#137365,#137366);
#109648=AXIS2_PLACEMENT_3D('',#250795,#137367,#137368);
#109649=AXIS2_PLACEMENT_3D('',#250808,#137369,#137370);
#109650=AXIS2_PLACEMENT_3D('',#250821,#137371,#137372);
#109651=AXIS2_PLACEMENT_3D('',#250822,#137373,#137374);
#109652=AXIS2_PLACEMENT_3D('',#250823,#137375,#137376);
#109653=AXIS2_PLACEMENT_3D('',#250824,#137377,#137378);
#109654=AXIS2_PLACEMENT_3D('',#250825,#137379,#137380);
#109655=AXIS2_PLACEMENT_3D('',#250838,#137381,#137382);
#109656=AXIS2_PLACEMENT_3D('',#250839,#137383,#137384);
#109657=AXIS2_PLACEMENT_3D('',#250840,#137385,#137386);
#109658=AXIS2_PLACEMENT_3D('',#250841,#137387,#137388);
#109659=AXIS2_PLACEMENT_3D('',#250842,#137389,#137390);
#109660=AXIS2_PLACEMENT_3D('',#250855,#137391,#137392);
#109661=AXIS2_PLACEMENT_3D('',#250856,#137393,#137394);
#109662=AXIS2_PLACEMENT_3D('',#250857,#137395,#137396);
#109663=AXIS2_PLACEMENT_3D('',#250858,#137397,#137398);
#109664=AXIS2_PLACEMENT_3D('',#250859,#137399,#137400);
#109665=AXIS2_PLACEMENT_3D('',#250872,#137401,#137402);
#109666=AXIS2_PLACEMENT_3D('',#250885,#137403,#137404);
#109667=AXIS2_PLACEMENT_3D('',#250886,#137405,#137406);
#109668=AXIS2_PLACEMENT_3D('',#250887,#137407,#137408);
#109669=AXIS2_PLACEMENT_3D('',#250888,#137409,#137410);
#109670=AXIS2_PLACEMENT_3D('',#250889,#137411,#137412);
#109671=AXIS2_PLACEMENT_3D('',#250908,#137413,#137414);
#109672=AXIS2_PLACEMENT_3D('',#250909,#137415,#137416);
#109673=AXIS2_PLACEMENT_3D('',#250910,#137417,#137418);
#109674=AXIS2_PLACEMENT_3D('',#250911,#137419,#137420);
#109675=AXIS2_PLACEMENT_3D('',#250912,#137421,#137422);
#109676=AXIS2_PLACEMENT_3D('',#250925,#137423,#137424);
#109677=AXIS2_PLACEMENT_3D('',#250944,#137425,#137426);
#109678=AXIS2_PLACEMENT_3D('',#250945,#137427,#137428);
#109679=AXIS2_PLACEMENT_3D('',#250946,#137429,#137430);
#109680=AXIS2_PLACEMENT_3D('',#250947,#137431,#137432);
#109681=AXIS2_PLACEMENT_3D('',#250948,#137433,#137434);
#109682=AXIS2_PLACEMENT_3D('',#250967,#137435,#137436);
#109683=AXIS2_PLACEMENT_3D('',#250980,#137437,#137438);
#109684=AXIS2_PLACEMENT_3D('',#250981,#137439,#137440);
#109685=AXIS2_PLACEMENT_3D('',#250982,#137441,#137442);
#109686=AXIS2_PLACEMENT_3D('',#250983,#137443,#137444);
#109687=AXIS2_PLACEMENT_3D('',#250984,#137445,#137446);
#109688=AXIS2_PLACEMENT_3D('',#251003,#137447,#137448);
#109689=AXIS2_PLACEMENT_3D('',#251004,#137449,#137450);
#109690=AXIS2_PLACEMENT_3D('',#251005,#137451,#137452);
#109691=AXIS2_PLACEMENT_3D('',#251006,#137453,#137454);
#109692=AXIS2_PLACEMENT_3D('',#251007,#137455,#137456);
#109693=AXIS2_PLACEMENT_3D('',#251020,#137457,#137458);
#109694=AXIS2_PLACEMENT_3D('',#251033,#137459,#137460);
#109695=AXIS2_PLACEMENT_3D('',#251034,#137461,#137462);
#109696=AXIS2_PLACEMENT_3D('',#251035,#137463,#137464);
#109697=AXIS2_PLACEMENT_3D('',#251036,#137465,#137466);
#109698=AXIS2_PLACEMENT_3D('',#251037,#137467,#137468);
#109699=AXIS2_PLACEMENT_3D('',#251050,#137469,#137470);
#109700=AXIS2_PLACEMENT_3D('',#251051,#137471,#137472);
#109701=AXIS2_PLACEMENT_3D('',#251052,#137473,#137474);
#109702=AXIS2_PLACEMENT_3D('',#251053,#137475,#137476);
#109703=AXIS2_PLACEMENT_3D('',#251054,#137477,#137478);
#109704=AXIS2_PLACEMENT_3D('',#251067,#137479,#137480);
#109705=AXIS2_PLACEMENT_3D('',#251068,#137481,#137482);
#109706=AXIS2_PLACEMENT_3D('',#251069,#137483,#137484);
#109707=AXIS2_PLACEMENT_3D('',#251070,#137485,#137486);
#109708=AXIS2_PLACEMENT_3D('',#251071,#137487,#137488);
#109709=AXIS2_PLACEMENT_3D('',#251084,#137489,#137490);
#109710=AXIS2_PLACEMENT_3D('',#251097,#137491,#137492);
#109711=AXIS2_PLACEMENT_3D('',#251098,#137493,#137494);
#109712=AXIS2_PLACEMENT_3D('',#251099,#137495,#137496);
#109713=AXIS2_PLACEMENT_3D('',#251100,#137497,#137498);
#109714=AXIS2_PLACEMENT_3D('',#251101,#137499,#137500);
#109715=AXIS2_PLACEMENT_3D('',#251120,#137501,#137502);
#109716=AXIS2_PLACEMENT_3D('',#251121,#137503,#137504);
#109717=AXIS2_PLACEMENT_3D('',#251122,#137505,#137506);
#109718=AXIS2_PLACEMENT_3D('',#251123,#137507,#137508);
#109719=AXIS2_PLACEMENT_3D('',#251124,#137509,#137510);
#109720=AXIS2_PLACEMENT_3D('',#251137,#137511,#137512);
#109721=AXIS2_PLACEMENT_3D('',#251156,#137513,#137514);
#109722=AXIS2_PLACEMENT_3D('',#251157,#137515,#137516);
#109723=AXIS2_PLACEMENT_3D('',#251158,#137517,#137518);
#109724=AXIS2_PLACEMENT_3D('',#251159,#137519,#137520);
#109725=AXIS2_PLACEMENT_3D('',#251160,#137521,#137522);
#109726=AXIS2_PLACEMENT_3D('',#251179,#137523,#137524);
#109727=AXIS2_PLACEMENT_3D('',#251192,#137525,#137526);
#109728=AXIS2_PLACEMENT_3D('',#251193,#137527,#137528);
#109729=AXIS2_PLACEMENT_3D('',#251194,#137529,#137530);
#109730=AXIS2_PLACEMENT_3D('',#251195,#137531,#137532);
#109731=AXIS2_PLACEMENT_3D('',#251196,#137533,#137534);
#109732=AXIS2_PLACEMENT_3D('',#251215,#137535,#137536);
#109733=AXIS2_PLACEMENT_3D('',#251216,#137537,#137538);
#109734=AXIS2_PLACEMENT_3D('',#251217,#137539,#137540);
#109735=AXIS2_PLACEMENT_3D('',#251218,#137541,#137542);
#109736=AXIS2_PLACEMENT_3D('',#251219,#137543,#137544);
#109737=AXIS2_PLACEMENT_3D('',#251232,#137545,#137546);
#109738=AXIS2_PLACEMENT_3D('',#251245,#137547,#137548);
#109739=AXIS2_PLACEMENT_3D('',#251246,#137549,#137550);
#109740=AXIS2_PLACEMENT_3D('',#251247,#137551,#137552);
#109741=AXIS2_PLACEMENT_3D('',#251248,#137553,#137554);
#109742=AXIS2_PLACEMENT_3D('',#251249,#137555,#137556);
#109743=AXIS2_PLACEMENT_3D('',#251262,#137557,#137558);
#109744=AXIS2_PLACEMENT_3D('',#251263,#137559,#137560);
#109745=AXIS2_PLACEMENT_3D('',#251264,#137561,#137562);
#109746=AXIS2_PLACEMENT_3D('',#251265,#137563,#137564);
#109747=AXIS2_PLACEMENT_3D('',#251266,#137565,#137566);
#109748=AXIS2_PLACEMENT_3D('',#251279,#137567,#137568);
#109749=AXIS2_PLACEMENT_3D('',#251280,#137569,#137570);
#109750=AXIS2_PLACEMENT_3D('',#251281,#137571,#137572);
#109751=AXIS2_PLACEMENT_3D('',#251282,#137573,#137574);
#109752=AXIS2_PLACEMENT_3D('',#251283,#137575,#137576);
#109753=AXIS2_PLACEMENT_3D('',#251296,#137577,#137578);
#109754=AXIS2_PLACEMENT_3D('',#251309,#137579,#137580);
#109755=AXIS2_PLACEMENT_3D('',#251310,#137581,#137582);
#109756=AXIS2_PLACEMENT_3D('',#251311,#137583,#137584);
#109757=AXIS2_PLACEMENT_3D('',#251312,#137585,#137586);
#109758=AXIS2_PLACEMENT_3D('',#251313,#137587,#137588);
#109759=AXIS2_PLACEMENT_3D('',#251332,#137589,#137590);
#109760=AXIS2_PLACEMENT_3D('',#251333,#137591,#137592);
#109761=AXIS2_PLACEMENT_3D('',#251334,#137593,#137594);
#109762=AXIS2_PLACEMENT_3D('',#251335,#137595,#137596);
#109763=AXIS2_PLACEMENT_3D('',#251336,#137597,#137598);
#109764=AXIS2_PLACEMENT_3D('',#251349,#137599,#137600);
#109765=AXIS2_PLACEMENT_3D('',#251368,#137601,#137602);
#109766=AXIS2_PLACEMENT_3D('',#251369,#137603,#137604);
#109767=AXIS2_PLACEMENT_3D('',#251370,#137605,#137606);
#109768=AXIS2_PLACEMENT_3D('',#251371,#137607,#137608);
#109769=AXIS2_PLACEMENT_3D('',#251372,#137609,#137610);
#109770=AXIS2_PLACEMENT_3D('',#251391,#137611,#137612);
#109771=AXIS2_PLACEMENT_3D('',#251404,#137613,#137614);
#109772=AXIS2_PLACEMENT_3D('',#251405,#137615,#137616);
#109773=AXIS2_PLACEMENT_3D('',#251406,#137617,#137618);
#109774=AXIS2_PLACEMENT_3D('',#251407,#137619,#137620);
#109775=AXIS2_PLACEMENT_3D('',#251408,#137621,#137622);
#109776=AXIS2_PLACEMENT_3D('',#251427,#137623,#137624);
#109777=AXIS2_PLACEMENT_3D('',#251428,#137625,#137626);
#109778=AXIS2_PLACEMENT_3D('',#251429,#137627,#137628);
#109779=AXIS2_PLACEMENT_3D('',#251430,#137629,#137630);
#109780=AXIS2_PLACEMENT_3D('',#251431,#137631,#137632);
#109781=AXIS2_PLACEMENT_3D('',#251444,#137633,#137634);
#109782=AXIS2_PLACEMENT_3D('',#251457,#137635,#137636);
#109783=AXIS2_PLACEMENT_3D('',#251458,#137637,#137638);
#109784=AXIS2_PLACEMENT_3D('',#251459,#137639,#137640);
#109785=AXIS2_PLACEMENT_3D('',#251460,#137641,#137642);
#109786=AXIS2_PLACEMENT_3D('',#251461,#137643,#137644);
#109787=AXIS2_PLACEMENT_3D('',#251474,#137645,#137646);
#109788=AXIS2_PLACEMENT_3D('',#251475,#137647,#137648);
#109789=AXIS2_PLACEMENT_3D('',#251476,#137649,#137650);
#109790=AXIS2_PLACEMENT_3D('',#251477,#137651,#137652);
#109791=AXIS2_PLACEMENT_3D('',#251478,#137653,#137654);
#109792=AXIS2_PLACEMENT_3D('',#251491,#137655,#137656);
#109793=AXIS2_PLACEMENT_3D('',#251492,#137657,#137658);
#109794=AXIS2_PLACEMENT_3D('',#251493,#137659,#137660);
#109795=AXIS2_PLACEMENT_3D('',#251494,#137661,#137662);
#109796=AXIS2_PLACEMENT_3D('',#251495,#137663,#137664);
#109797=AXIS2_PLACEMENT_3D('',#251508,#137665,#137666);
#109798=AXIS2_PLACEMENT_3D('',#251521,#137667,#137668);
#109799=AXIS2_PLACEMENT_3D('',#251522,#137669,#137670);
#109800=AXIS2_PLACEMENT_3D('',#251523,#137671,#137672);
#109801=AXIS2_PLACEMENT_3D('',#251524,#137673,#137674);
#109802=AXIS2_PLACEMENT_3D('',#251525,#137675,#137676);
#109803=AXIS2_PLACEMENT_3D('',#251544,#137677,#137678);
#109804=AXIS2_PLACEMENT_3D('',#251545,#137679,#137680);
#109805=AXIS2_PLACEMENT_3D('',#251546,#137681,#137682);
#109806=AXIS2_PLACEMENT_3D('',#251547,#137683,#137684);
#109807=AXIS2_PLACEMENT_3D('',#251548,#137685,#137686);
#109808=AXIS2_PLACEMENT_3D('',#251561,#137687,#137688);
#109809=AXIS2_PLACEMENT_3D('',#251580,#137689,#137690);
#109810=AXIS2_PLACEMENT_3D('',#251581,#137691,#137692);
#109811=AXIS2_PLACEMENT_3D('',#251582,#137693,#137694);
#109812=AXIS2_PLACEMENT_3D('',#251583,#137695,#137696);
#109813=AXIS2_PLACEMENT_3D('',#251584,#137697,#137698);
#109814=AXIS2_PLACEMENT_3D('',#251603,#137699,#137700);
#109815=AXIS2_PLACEMENT_3D('',#251616,#137701,#137702);
#109816=AXIS2_PLACEMENT_3D('',#251617,#137703,#137704);
#109817=AXIS2_PLACEMENT_3D('',#251618,#137705,#137706);
#109818=AXIS2_PLACEMENT_3D('',#251619,#137707,#137708);
#109819=AXIS2_PLACEMENT_3D('',#251620,#137709,#137710);
#109820=AXIS2_PLACEMENT_3D('',#251639,#137711,#137712);
#109821=AXIS2_PLACEMENT_3D('',#251640,#137713,#137714);
#109822=AXIS2_PLACEMENT_3D('',#251641,#137715,#137716);
#109823=AXIS2_PLACEMENT_3D('',#251642,#137717,#137718);
#109824=AXIS2_PLACEMENT_3D('',#251643,#137719,#137720);
#109825=AXIS2_PLACEMENT_3D('',#251656,#137721,#137722);
#109826=AXIS2_PLACEMENT_3D('',#251669,#137723,#137724);
#109827=AXIS2_PLACEMENT_3D('',#251670,#137725,#137726);
#109828=AXIS2_PLACEMENT_3D('',#251671,#137727,#137728);
#109829=AXIS2_PLACEMENT_3D('',#251672,#137729,#137730);
#109830=AXIS2_PLACEMENT_3D('',#251673,#137731,#137732);
#109831=AXIS2_PLACEMENT_3D('',#251686,#137733,#137734);
#109832=AXIS2_PLACEMENT_3D('',#251687,#137735,#137736);
#109833=AXIS2_PLACEMENT_3D('',#251688,#137737,#137738);
#109834=AXIS2_PLACEMENT_3D('',#251689,#137739,#137740);
#109835=AXIS2_PLACEMENT_3D('',#251690,#137741,#137742);
#109836=AXIS2_PLACEMENT_3D('',#251703,#137743,#137744);
#109837=AXIS2_PLACEMENT_3D('',#251704,#137745,#137746);
#109838=AXIS2_PLACEMENT_3D('',#251705,#137747,#137748);
#109839=AXIS2_PLACEMENT_3D('',#251706,#137749,#137750);
#109840=AXIS2_PLACEMENT_3D('',#251707,#137751,#137752);
#109841=AXIS2_PLACEMENT_3D('',#251720,#137753,#137754);
#109842=AXIS2_PLACEMENT_3D('',#251733,#137755,#137756);
#109843=AXIS2_PLACEMENT_3D('',#251734,#137757,#137758);
#109844=AXIS2_PLACEMENT_3D('',#251735,#137759,#137760);
#109845=AXIS2_PLACEMENT_3D('',#251736,#137761,#137762);
#109846=AXIS2_PLACEMENT_3D('',#251737,#137763,#137764);
#109847=AXIS2_PLACEMENT_3D('',#251756,#137765,#137766);
#109848=AXIS2_PLACEMENT_3D('',#251757,#137767,#137768);
#109849=AXIS2_PLACEMENT_3D('',#251758,#137769,#137770);
#109850=AXIS2_PLACEMENT_3D('',#251759,#137771,#137772);
#109851=AXIS2_PLACEMENT_3D('',#251760,#137773,#137774);
#109852=AXIS2_PLACEMENT_3D('',#251773,#137775,#137776);
#109853=AXIS2_PLACEMENT_3D('',#251792,#137777,#137778);
#109854=AXIS2_PLACEMENT_3D('',#251793,#137779,#137780);
#109855=AXIS2_PLACEMENT_3D('',#251794,#137781,#137782);
#109856=AXIS2_PLACEMENT_3D('',#251795,#137783,#137784);
#109857=AXIS2_PLACEMENT_3D('',#251796,#137785,#137786);
#109858=AXIS2_PLACEMENT_3D('',#251815,#137787,#137788);
#109859=AXIS2_PLACEMENT_3D('',#251828,#137789,#137790);
#109860=AXIS2_PLACEMENT_3D('',#251829,#137791,#137792);
#109861=AXIS2_PLACEMENT_3D('',#251830,#137793,#137794);
#109862=AXIS2_PLACEMENT_3D('',#251831,#137795,#137796);
#109863=AXIS2_PLACEMENT_3D('',#251832,#137797,#137798);
#109864=AXIS2_PLACEMENT_3D('',#251851,#137799,#137800);
#109865=AXIS2_PLACEMENT_3D('',#251852,#137801,#137802);
#109866=AXIS2_PLACEMENT_3D('',#251853,#137803,#137804);
#109867=AXIS2_PLACEMENT_3D('',#251854,#137805,#137806);
#109868=AXIS2_PLACEMENT_3D('',#251855,#137807,#137808);
#109869=AXIS2_PLACEMENT_3D('',#251868,#137809,#137810);
#109870=AXIS2_PLACEMENT_3D('',#251881,#137811,#137812);
#109871=AXIS2_PLACEMENT_3D('',#251882,#137813,#137814);
#109872=AXIS2_PLACEMENT_3D('',#251883,#137815,#137816);
#109873=AXIS2_PLACEMENT_3D('',#251884,#137817,#137818);
#109874=AXIS2_PLACEMENT_3D('',#251885,#137819,#137820);
#109875=AXIS2_PLACEMENT_3D('',#251898,#137821,#137822);
#109876=AXIS2_PLACEMENT_3D('',#251899,#137823,#137824);
#109877=AXIS2_PLACEMENT_3D('',#251900,#137825,#137826);
#109878=AXIS2_PLACEMENT_3D('',#251901,#137827,#137828);
#109879=AXIS2_PLACEMENT_3D('',#251902,#137829,#137830);
#109880=AXIS2_PLACEMENT_3D('',#251915,#137831,#137832);
#109881=AXIS2_PLACEMENT_3D('',#251916,#137833,#137834);
#109882=AXIS2_PLACEMENT_3D('',#251917,#137835,#137836);
#109883=AXIS2_PLACEMENT_3D('',#251918,#137837,#137838);
#109884=AXIS2_PLACEMENT_3D('',#251919,#137839,#137840);
#109885=AXIS2_PLACEMENT_3D('',#251932,#137841,#137842);
#109886=AXIS2_PLACEMENT_3D('',#251945,#137843,#137844);
#109887=AXIS2_PLACEMENT_3D('',#251946,#137845,#137846);
#109888=AXIS2_PLACEMENT_3D('',#251947,#137847,#137848);
#109889=AXIS2_PLACEMENT_3D('',#251948,#137849,#137850);
#109890=AXIS2_PLACEMENT_3D('',#251949,#137851,#137852);
#109891=AXIS2_PLACEMENT_3D('',#251968,#137853,#137854);
#109892=AXIS2_PLACEMENT_3D('',#251969,#137855,#137856);
#109893=AXIS2_PLACEMENT_3D('',#251970,#137857,#137858);
#109894=AXIS2_PLACEMENT_3D('',#251971,#137859,#137860);
#109895=AXIS2_PLACEMENT_3D('',#251972,#137861,#137862);
#109896=AXIS2_PLACEMENT_3D('',#251985,#137863,#137864);
#109897=AXIS2_PLACEMENT_3D('',#252004,#137865,#137866);
#109898=AXIS2_PLACEMENT_3D('',#252005,#137867,#137868);
#109899=AXIS2_PLACEMENT_3D('',#252006,#137869,#137870);
#109900=AXIS2_PLACEMENT_3D('',#252007,#137871,#137872);
#109901=AXIS2_PLACEMENT_3D('',#252008,#137873,#137874);
#109902=AXIS2_PLACEMENT_3D('',#252027,#137875,#137876);
#109903=AXIS2_PLACEMENT_3D('',#252040,#137877,#137878);
#109904=AXIS2_PLACEMENT_3D('',#252041,#137879,#137880);
#109905=AXIS2_PLACEMENT_3D('',#252042,#137881,#137882);
#109906=AXIS2_PLACEMENT_3D('',#252043,#137883,#137884);
#109907=AXIS2_PLACEMENT_3D('',#252044,#137885,#137886);
#109908=AXIS2_PLACEMENT_3D('',#252063,#137887,#137888);
#109909=AXIS2_PLACEMENT_3D('',#252064,#137889,#137890);
#109910=AXIS2_PLACEMENT_3D('',#252065,#137891,#137892);
#109911=AXIS2_PLACEMENT_3D('',#252066,#137893,#137894);
#109912=AXIS2_PLACEMENT_3D('',#252067,#137895,#137896);
#109913=AXIS2_PLACEMENT_3D('',#252080,#137897,#137898);
#109914=AXIS2_PLACEMENT_3D('',#252093,#137899,#137900);
#109915=AXIS2_PLACEMENT_3D('',#252094,#137901,#137902);
#109916=AXIS2_PLACEMENT_3D('',#252095,#137903,#137904);
#109917=AXIS2_PLACEMENT_3D('',#252096,#137905,#137906);
#109918=AXIS2_PLACEMENT_3D('',#252097,#137907,#137908);
#109919=AXIS2_PLACEMENT_3D('',#252110,#137909,#137910);
#109920=AXIS2_PLACEMENT_3D('',#252111,#137911,#137912);
#109921=AXIS2_PLACEMENT_3D('',#252112,#137913,#137914);
#109922=AXIS2_PLACEMENT_3D('',#252113,#137915,#137916);
#109923=AXIS2_PLACEMENT_3D('',#252114,#137917,#137918);
#109924=AXIS2_PLACEMENT_3D('',#252127,#137919,#137920);
#109925=AXIS2_PLACEMENT_3D('',#252128,#137921,#137922);
#109926=AXIS2_PLACEMENT_3D('',#252129,#137923,#137924);
#109927=AXIS2_PLACEMENT_3D('',#252130,#137925,#137926);
#109928=AXIS2_PLACEMENT_3D('',#252131,#137927,#137928);
#109929=AXIS2_PLACEMENT_3D('',#252144,#137929,#137930);
#109930=AXIS2_PLACEMENT_3D('',#252157,#137931,#137932);
#109931=AXIS2_PLACEMENT_3D('',#252158,#137933,#137934);
#109932=AXIS2_PLACEMENT_3D('',#252159,#137935,#137936);
#109933=AXIS2_PLACEMENT_3D('',#252160,#137937,#137938);
#109934=AXIS2_PLACEMENT_3D('',#252161,#137939,#137940);
#109935=AXIS2_PLACEMENT_3D('',#252180,#137941,#137942);
#109936=AXIS2_PLACEMENT_3D('',#252181,#137943,#137944);
#109937=AXIS2_PLACEMENT_3D('',#252182,#137945,#137946);
#109938=AXIS2_PLACEMENT_3D('',#252183,#137947,#137948);
#109939=AXIS2_PLACEMENT_3D('',#252184,#137949,#137950);
#109940=AXIS2_PLACEMENT_3D('',#252197,#137951,#137952);
#109941=AXIS2_PLACEMENT_3D('',#252216,#137953,#137954);
#109942=AXIS2_PLACEMENT_3D('',#252217,#137955,#137956);
#109943=AXIS2_PLACEMENT_3D('',#252218,#137957,#137958);
#109944=AXIS2_PLACEMENT_3D('',#252219,#137959,#137960);
#109945=AXIS2_PLACEMENT_3D('',#252220,#137961,#137962);
#109946=AXIS2_PLACEMENT_3D('',#252239,#137963,#137964);
#109947=AXIS2_PLACEMENT_3D('',#252252,#137965,#137966);
#109948=AXIS2_PLACEMENT_3D('',#252253,#137967,#137968);
#109949=AXIS2_PLACEMENT_3D('',#252254,#137969,#137970);
#109950=AXIS2_PLACEMENT_3D('',#252255,#137971,#137972);
#109951=AXIS2_PLACEMENT_3D('',#252256,#137973,#137974);
#109952=AXIS2_PLACEMENT_3D('',#252275,#137975,#137976);
#109953=AXIS2_PLACEMENT_3D('',#252276,#137977,#137978);
#109954=AXIS2_PLACEMENT_3D('',#252277,#137979,#137980);
#109955=AXIS2_PLACEMENT_3D('',#252278,#137981,#137982);
#109956=AXIS2_PLACEMENT_3D('',#252279,#137983,#137984);
#109957=AXIS2_PLACEMENT_3D('',#252292,#137985,#137986);
#109958=AXIS2_PLACEMENT_3D('',#252305,#137987,#137988);
#109959=AXIS2_PLACEMENT_3D('',#252306,#137989,#137990);
#109960=AXIS2_PLACEMENT_3D('',#252307,#137991,#137992);
#109961=AXIS2_PLACEMENT_3D('',#252308,#137993,#137994);
#109962=AXIS2_PLACEMENT_3D('',#252309,#137995,#137996);
#109963=AXIS2_PLACEMENT_3D('',#252322,#137997,#137998);
#109964=AXIS2_PLACEMENT_3D('',#252323,#137999,#138000);
#109965=AXIS2_PLACEMENT_3D('',#252324,#138001,#138002);
#109966=AXIS2_PLACEMENT_3D('',#252325,#138003,#138004);
#109967=AXIS2_PLACEMENT_3D('',#252326,#138005,#138006);
#109968=AXIS2_PLACEMENT_3D('',#252339,#138007,#138008);
#109969=AXIS2_PLACEMENT_3D('',#252340,#138009,#138010);
#109970=AXIS2_PLACEMENT_3D('',#252341,#138011,#138012);
#109971=AXIS2_PLACEMENT_3D('',#252342,#138013,#138014);
#109972=AXIS2_PLACEMENT_3D('',#252343,#138015,#138016);
#109973=AXIS2_PLACEMENT_3D('',#252356,#138017,#138018);
#109974=AXIS2_PLACEMENT_3D('',#252369,#138019,#138020);
#109975=AXIS2_PLACEMENT_3D('',#252370,#138021,#138022);
#109976=AXIS2_PLACEMENT_3D('',#252371,#138023,#138024);
#109977=AXIS2_PLACEMENT_3D('',#252372,#138025,#138026);
#109978=AXIS2_PLACEMENT_3D('',#252373,#138027,#138028);
#109979=AXIS2_PLACEMENT_3D('',#252392,#138029,#138030);
#109980=AXIS2_PLACEMENT_3D('',#252393,#138031,#138032);
#109981=AXIS2_PLACEMENT_3D('',#252394,#138033,#138034);
#109982=AXIS2_PLACEMENT_3D('',#252395,#138035,#138036);
#109983=AXIS2_PLACEMENT_3D('',#252396,#138037,#138038);
#109984=AXIS2_PLACEMENT_3D('',#252409,#138039,#138040);
#109985=AXIS2_PLACEMENT_3D('',#252428,#138041,#138042);
#109986=AXIS2_PLACEMENT_3D('',#252429,#138043,#138044);
#109987=AXIS2_PLACEMENT_3D('',#252430,#138045,#138046);
#109988=AXIS2_PLACEMENT_3D('',#252431,#138047,#138048);
#109989=AXIS2_PLACEMENT_3D('',#252432,#138049,#138050);
#109990=AXIS2_PLACEMENT_3D('',#252451,#138051,#138052);
#109991=AXIS2_PLACEMENT_3D('',#252464,#138053,#138054);
#109992=AXIS2_PLACEMENT_3D('',#252465,#138055,#138056);
#109993=AXIS2_PLACEMENT_3D('',#252466,#138057,#138058);
#109994=AXIS2_PLACEMENT_3D('',#252467,#138059,#138060);
#109995=AXIS2_PLACEMENT_3D('',#252468,#138061,#138062);
#109996=AXIS2_PLACEMENT_3D('',#252487,#138063,#138064);
#109997=AXIS2_PLACEMENT_3D('',#252488,#138065,#138066);
#109998=AXIS2_PLACEMENT_3D('',#252489,#138067,#138068);
#109999=AXIS2_PLACEMENT_3D('',#252490,#138069,#138070);
#110000=AXIS2_PLACEMENT_3D('',#252491,#138071,#138072);
#110001=AXIS2_PLACEMENT_3D('',#252504,#138073,#138074);
#110002=AXIS2_PLACEMENT_3D('',#252517,#138075,#138076);
#110003=AXIS2_PLACEMENT_3D('',#252518,#138077,#138078);
#110004=AXIS2_PLACEMENT_3D('',#252519,#138079,#138080);
#110005=AXIS2_PLACEMENT_3D('',#252520,#138081,#138082);
#110006=AXIS2_PLACEMENT_3D('',#252521,#138083,#138084);
#110007=AXIS2_PLACEMENT_3D('',#252534,#138085,#138086);
#110008=AXIS2_PLACEMENT_3D('',#252535,#138087,#138088);
#110009=AXIS2_PLACEMENT_3D('',#252536,#138089,#138090);
#110010=AXIS2_PLACEMENT_3D('',#252537,#138091,#138092);
#110011=AXIS2_PLACEMENT_3D('',#252538,#138093,#138094);
#110012=AXIS2_PLACEMENT_3D('',#252551,#138095,#138096);
#110013=AXIS2_PLACEMENT_3D('',#252552,#138097,#138098);
#110014=AXIS2_PLACEMENT_3D('',#252553,#138099,#138100);
#110015=AXIS2_PLACEMENT_3D('',#252554,#138101,#138102);
#110016=AXIS2_PLACEMENT_3D('',#252555,#138103,#138104);
#110017=AXIS2_PLACEMENT_3D('',#252568,#138105,#138106);
#110018=AXIS2_PLACEMENT_3D('',#252581,#138107,#138108);
#110019=AXIS2_PLACEMENT_3D('',#252582,#138109,#138110);
#110020=AXIS2_PLACEMENT_3D('',#252583,#138111,#138112);
#110021=AXIS2_PLACEMENT_3D('',#252584,#138113,#138114);
#110022=AXIS2_PLACEMENT_3D('',#252585,#138115,#138116);
#110023=AXIS2_PLACEMENT_3D('',#252604,#138117,#138118);
#110024=AXIS2_PLACEMENT_3D('',#252605,#138119,#138120);
#110025=AXIS2_PLACEMENT_3D('',#252606,#138121,#138122);
#110026=AXIS2_PLACEMENT_3D('',#252607,#138123,#138124);
#110027=AXIS2_PLACEMENT_3D('',#252608,#138125,#138126);
#110028=AXIS2_PLACEMENT_3D('',#252621,#138127,#138128);
#110029=AXIS2_PLACEMENT_3D('',#252640,#138129,#138130);
#110030=AXIS2_PLACEMENT_3D('',#252641,#138131,#138132);
#110031=AXIS2_PLACEMENT_3D('',#252642,#138133,#138134);
#110032=AXIS2_PLACEMENT_3D('',#252643,#138135,#138136);
#110033=AXIS2_PLACEMENT_3D('',#252644,#138137,#138138);
#110034=AXIS2_PLACEMENT_3D('',#252663,#138139,#138140);
#110035=AXIS2_PLACEMENT_3D('',#252676,#138141,#138142);
#110036=AXIS2_PLACEMENT_3D('',#252677,#138143,#138144);
#110037=AXIS2_PLACEMENT_3D('',#252678,#138145,#138146);
#110038=AXIS2_PLACEMENT_3D('',#252679,#138147,#138148);
#110039=AXIS2_PLACEMENT_3D('',#252680,#138149,#138150);
#110040=AXIS2_PLACEMENT_3D('',#252699,#138151,#138152);
#110041=AXIS2_PLACEMENT_3D('',#252700,#138153,#138154);
#110042=AXIS2_PLACEMENT_3D('',#252701,#138155,#138156);
#110043=AXIS2_PLACEMENT_3D('',#252702,#138157,#138158);
#110044=AXIS2_PLACEMENT_3D('',#252703,#138159,#138160);
#110045=AXIS2_PLACEMENT_3D('',#252716,#138161,#138162);
#110046=AXIS2_PLACEMENT_3D('',#252729,#138163,#138164);
#110047=AXIS2_PLACEMENT_3D('',#252730,#138165,#138166);
#110048=AXIS2_PLACEMENT_3D('',#252731,#138167,#138168);
#110049=AXIS2_PLACEMENT_3D('',#252732,#138169,#138170);
#110050=AXIS2_PLACEMENT_3D('',#252733,#138171,#138172);
#110051=AXIS2_PLACEMENT_3D('',#252746,#138173,#138174);
#110052=AXIS2_PLACEMENT_3D('',#252747,#138175,#138176);
#110053=AXIS2_PLACEMENT_3D('',#252748,#138177,#138178);
#110054=AXIS2_PLACEMENT_3D('',#252749,#138179,#138180);
#110055=AXIS2_PLACEMENT_3D('',#252750,#138181,#138182);
#110056=AXIS2_PLACEMENT_3D('',#252763,#138183,#138184);
#110057=AXIS2_PLACEMENT_3D('',#252764,#138185,#138186);
#110058=AXIS2_PLACEMENT_3D('',#252765,#138187,#138188);
#110059=AXIS2_PLACEMENT_3D('',#252766,#138189,#138190);
#110060=AXIS2_PLACEMENT_3D('',#252767,#138191,#138192);
#110061=AXIS2_PLACEMENT_3D('',#252780,#138193,#138194);
#110062=AXIS2_PLACEMENT_3D('',#252793,#138195,#138196);
#110063=AXIS2_PLACEMENT_3D('',#252794,#138197,#138198);
#110064=AXIS2_PLACEMENT_3D('',#252795,#138199,#138200);
#110065=AXIS2_PLACEMENT_3D('',#252796,#138201,#138202);
#110066=AXIS2_PLACEMENT_3D('',#252797,#138203,#138204);
#110067=AXIS2_PLACEMENT_3D('',#252816,#138205,#138206);
#110068=AXIS2_PLACEMENT_3D('',#252817,#138207,#138208);
#110069=AXIS2_PLACEMENT_3D('',#252818,#138209,#138210);
#110070=AXIS2_PLACEMENT_3D('',#252819,#138211,#138212);
#110071=AXIS2_PLACEMENT_3D('',#252820,#138213,#138214);
#110072=AXIS2_PLACEMENT_3D('',#252833,#138215,#138216);
#110073=AXIS2_PLACEMENT_3D('',#252852,#138217,#138218);
#110074=AXIS2_PLACEMENT_3D('',#252853,#138219,#138220);
#110075=AXIS2_PLACEMENT_3D('',#252854,#138221,#138222);
#110076=AXIS2_PLACEMENT_3D('',#252855,#138223,#138224);
#110077=AXIS2_PLACEMENT_3D('',#252856,#138225,#138226);
#110078=AXIS2_PLACEMENT_3D('',#252875,#138227,#138228);
#110079=AXIS2_PLACEMENT_3D('',#252888,#138229,#138230);
#110080=AXIS2_PLACEMENT_3D('',#252889,#138231,#138232);
#110081=AXIS2_PLACEMENT_3D('',#252890,#138233,#138234);
#110082=AXIS2_PLACEMENT_3D('',#252891,#138235,#138236);
#110083=AXIS2_PLACEMENT_3D('',#252892,#138237,#138238);
#110084=AXIS2_PLACEMENT_3D('',#252911,#138239,#138240);
#110085=AXIS2_PLACEMENT_3D('',#252912,#138241,#138242);
#110086=AXIS2_PLACEMENT_3D('',#252913,#138243,#138244);
#110087=AXIS2_PLACEMENT_3D('',#252914,#138245,#138246);
#110088=AXIS2_PLACEMENT_3D('',#252915,#138247,#138248);
#110089=AXIS2_PLACEMENT_3D('',#252928,#138249,#138250);
#110090=AXIS2_PLACEMENT_3D('',#252941,#138251,#138252);
#110091=AXIS2_PLACEMENT_3D('',#252942,#138253,#138254);
#110092=AXIS2_PLACEMENT_3D('',#252943,#138255,#138256);
#110093=AXIS2_PLACEMENT_3D('',#252944,#138257,#138258);
#110094=AXIS2_PLACEMENT_3D('',#252945,#138259,#138260);
#110095=AXIS2_PLACEMENT_3D('',#252958,#138261,#138262);
#110096=AXIS2_PLACEMENT_3D('',#252959,#138263,#138264);
#110097=AXIS2_PLACEMENT_3D('',#252960,#138265,#138266);
#110098=AXIS2_PLACEMENT_3D('',#252961,#138267,#138268);
#110099=AXIS2_PLACEMENT_3D('',#252962,#138269,#138270);
#110100=AXIS2_PLACEMENT_3D('',#252975,#138271,#138272);
#110101=AXIS2_PLACEMENT_3D('',#252976,#138273,#138274);
#110102=AXIS2_PLACEMENT_3D('',#252977,#138275,#138276);
#110103=AXIS2_PLACEMENT_3D('',#252978,#138277,#138278);
#110104=AXIS2_PLACEMENT_3D('',#252979,#138279,#138280);
#110105=AXIS2_PLACEMENT_3D('',#252992,#138281,#138282);
#110106=AXIS2_PLACEMENT_3D('',#253005,#138283,#138284);
#110107=AXIS2_PLACEMENT_3D('',#253006,#138285,#138286);
#110108=AXIS2_PLACEMENT_3D('',#253007,#138287,#138288);
#110109=AXIS2_PLACEMENT_3D('',#253008,#138289,#138290);
#110110=AXIS2_PLACEMENT_3D('',#253009,#138291,#138292);
#110111=AXIS2_PLACEMENT_3D('',#253028,#138293,#138294);
#110112=AXIS2_PLACEMENT_3D('',#253029,#138295,#138296);
#110113=AXIS2_PLACEMENT_3D('',#253030,#138297,#138298);
#110114=AXIS2_PLACEMENT_3D('',#253031,#138299,#138300);
#110115=AXIS2_PLACEMENT_3D('',#253032,#138301,#138302);
#110116=AXIS2_PLACEMENT_3D('',#253045,#138303,#138304);
#110117=AXIS2_PLACEMENT_3D('',#253064,#138305,#138306);
#110118=AXIS2_PLACEMENT_3D('',#253065,#138307,#138308);
#110119=AXIS2_PLACEMENT_3D('',#253066,#138309,#138310);
#110120=AXIS2_PLACEMENT_3D('',#253067,#138311,#138312);
#110121=AXIS2_PLACEMENT_3D('',#253068,#138313,#138314);
#110122=AXIS2_PLACEMENT_3D('',#253087,#138315,#138316);
#110123=AXIS2_PLACEMENT_3D('',#253100,#138317,#138318);
#110124=AXIS2_PLACEMENT_3D('',#253101,#138319,#138320);
#110125=AXIS2_PLACEMENT_3D('',#253102,#138321,#138322);
#110126=AXIS2_PLACEMENT_3D('',#253103,#138323,#138324);
#110127=AXIS2_PLACEMENT_3D('',#253104,#138325,#138326);
#110128=AXIS2_PLACEMENT_3D('',#253123,#138327,#138328);
#110129=AXIS2_PLACEMENT_3D('',#253124,#138329,#138330);
#110130=AXIS2_PLACEMENT_3D('',#253125,#138331,#138332);
#110131=AXIS2_PLACEMENT_3D('',#253126,#138333,#138334);
#110132=AXIS2_PLACEMENT_3D('',#253127,#138335,#138336);
#110133=AXIS2_PLACEMENT_3D('',#253140,#138337,#138338);
#110134=AXIS2_PLACEMENT_3D('',#253153,#138339,#138340);
#110135=AXIS2_PLACEMENT_3D('',#253154,#138341,#138342);
#110136=AXIS2_PLACEMENT_3D('',#253155,#138343,#138344);
#110137=AXIS2_PLACEMENT_3D('',#253156,#138345,#138346);
#110138=AXIS2_PLACEMENT_3D('',#253157,#138347,#138348);
#110139=AXIS2_PLACEMENT_3D('',#253170,#138349,#138350);
#110140=AXIS2_PLACEMENT_3D('',#253171,#138351,#138352);
#110141=AXIS2_PLACEMENT_3D('',#253172,#138353,#138354);
#110142=AXIS2_PLACEMENT_3D('',#253173,#138355,#138356);
#110143=AXIS2_PLACEMENT_3D('',#253174,#138357,#138358);
#110144=AXIS2_PLACEMENT_3D('',#253187,#138359,#138360);
#110145=AXIS2_PLACEMENT_3D('',#253188,#138361,#138362);
#110146=AXIS2_PLACEMENT_3D('',#253189,#138363,#138364);
#110147=AXIS2_PLACEMENT_3D('',#253190,#138365,#138366);
#110148=AXIS2_PLACEMENT_3D('',#253191,#138367,#138368);
#110149=AXIS2_PLACEMENT_3D('',#253204,#138369,#138370);
#110150=AXIS2_PLACEMENT_3D('',#253217,#138371,#138372);
#110151=AXIS2_PLACEMENT_3D('',#253218,#138373,#138374);
#110152=AXIS2_PLACEMENT_3D('',#253219,#138375,#138376);
#110153=AXIS2_PLACEMENT_3D('',#253220,#138377,#138378);
#110154=AXIS2_PLACEMENT_3D('',#253221,#138379,#138380);
#110155=AXIS2_PLACEMENT_3D('',#253240,#138381,#138382);
#110156=AXIS2_PLACEMENT_3D('',#253241,#138383,#138384);
#110157=AXIS2_PLACEMENT_3D('',#253242,#138385,#138386);
#110158=AXIS2_PLACEMENT_3D('',#253243,#138387,#138388);
#110159=AXIS2_PLACEMENT_3D('',#253244,#138389,#138390);
#110160=AXIS2_PLACEMENT_3D('',#253257,#138391,#138392);
#110161=AXIS2_PLACEMENT_3D('',#253276,#138393,#138394);
#110162=AXIS2_PLACEMENT_3D('',#253277,#138395,#138396);
#110163=AXIS2_PLACEMENT_3D('',#253278,#138397,#138398);
#110164=AXIS2_PLACEMENT_3D('',#253279,#138399,#138400);
#110165=AXIS2_PLACEMENT_3D('',#253280,#138401,#138402);
#110166=AXIS2_PLACEMENT_3D('',#253299,#138403,#138404);
#110167=AXIS2_PLACEMENT_3D('',#253312,#138405,#138406);
#110168=AXIS2_PLACEMENT_3D('',#253313,#138407,#138408);
#110169=AXIS2_PLACEMENT_3D('',#253314,#138409,#138410);
#110170=AXIS2_PLACEMENT_3D('',#253315,#138411,#138412);
#110171=AXIS2_PLACEMENT_3D('',#253316,#138413,#138414);
#110172=AXIS2_PLACEMENT_3D('',#253335,#138415,#138416);
#110173=AXIS2_PLACEMENT_3D('',#253336,#138417,#138418);
#110174=AXIS2_PLACEMENT_3D('',#253337,#138419,#138420);
#110175=AXIS2_PLACEMENT_3D('',#253338,#138421,#138422);
#110176=AXIS2_PLACEMENT_3D('',#253339,#138423,#138424);
#110177=AXIS2_PLACEMENT_3D('',#253352,#138425,#138426);
#110178=AXIS2_PLACEMENT_3D('',#253365,#138427,#138428);
#110179=AXIS2_PLACEMENT_3D('',#253366,#138429,#138430);
#110180=AXIS2_PLACEMENT_3D('',#253367,#138431,#138432);
#110181=AXIS2_PLACEMENT_3D('',#253368,#138433,#138434);
#110182=AXIS2_PLACEMENT_3D('',#253369,#138435,#138436);
#110183=AXIS2_PLACEMENT_3D('',#253382,#138437,#138438);
#110184=AXIS2_PLACEMENT_3D('',#253383,#138439,#138440);
#110185=AXIS2_PLACEMENT_3D('',#253384,#138441,#138442);
#110186=AXIS2_PLACEMENT_3D('',#253386,#138443,#138444);
#110187=AXIS2_PLACEMENT_3D('',#253388,#138445,#138446);
#110188=AXIS2_PLACEMENT_3D('',#253389,#138447,#138448);
#110189=AXIS2_PLACEMENT_3D('',#253390,#138449,#138450);
#110190=AXIS2_PLACEMENT_3D('',#253392,#138451,#138452);
#110191=AXIS2_PLACEMENT_3D('',#253394,#138453,#138454);
#110192=AXIS2_PLACEMENT_3D('',#253395,#138455,#138456);
#110193=AXIS2_PLACEMENT_3D('',#253396,#138457,#138458);
#110194=AXIS2_PLACEMENT_3D('',#253398,#138459,#138460);
#110195=AXIS2_PLACEMENT_3D('',#253400,#138461,#138462);
#110196=AXIS2_PLACEMENT_3D('',#253402,#138463,#138464);
#110197=AXIS2_PLACEMENT_3D('',#253403,#138465,#138466);
#110198=AXIS2_PLACEMENT_3D('',#253404,#138467,#138468);
#110199=AXIS2_PLACEMENT_3D('',#253406,#138469,#138470);
#110200=AXIS2_PLACEMENT_3D('',#253408,#138472,#138473);
#110201=AXIS2_PLACEMENT_3D('',#253410,#138475,#138476);
#110202=AXIS2_PLACEMENT_3D('',#253412,#138477,#138478);
#110203=AXIS2_PLACEMENT_3D('',#253415,#138480,#138481);
#110204=AXIS2_PLACEMENT_3D('',#253416,#138482,#138483);
#110205=AXIS2_PLACEMENT_3D('',#253417,#138484,#138485);
#110206=AXIS2_PLACEMENT_3D('',#253418,#138486,#138487);
#110207=AXIS2_PLACEMENT_3D('',#253419,#138488,#138489);
#110208=AXIS2_PLACEMENT_3D('',#253421,#138490,#138491);
#110209=AXIS2_PLACEMENT_3D('',#253423,#138492,#138493);
#110210=AXIS2_PLACEMENT_3D('',#253424,#138494,#138495);
#110211=AXIS2_PLACEMENT_3D('',#253425,#138496,#138497);
#110212=AXIS2_PLACEMENT_3D('',#253427,#138498,#138499);
#110213=AXIS2_PLACEMENT_3D('',#253429,#138500,#138501);
#110214=AXIS2_PLACEMENT_3D('',#253430,#138502,#138503);
#110215=AXIS2_PLACEMENT_3D('',#253431,#138504,#138505);
#110216=AXIS2_PLACEMENT_3D('',#253433,#138506,#138507);
#110217=AXIS2_PLACEMENT_3D('',#253435,#138509,#138510);
#110218=AXIS2_PLACEMENT_3D('',#253438,#138512,#138513);
#110219=AXIS2_PLACEMENT_3D('',#253439,#138514,#138515);
#110220=AXIS2_PLACEMENT_3D('',#253440,#138516,#138517);
#110221=AXIS2_PLACEMENT_3D('',#253441,#138518,#138519);
#110222=AXIS2_PLACEMENT_3D('',#253443,#138520,#138521);
#110223=AXIS2_PLACEMENT_3D('',#253445,#138522,#138523);
#110224=AXIS2_PLACEMENT_3D('',#253446,#138524,#138525);
#110225=AXIS2_PLACEMENT_3D('',#253447,#138526,#138527);
#110226=AXIS2_PLACEMENT_3D('',#253450,#138528,#138529);
#110227=AXIS2_PLACEMENT_3D('',#253452,#138530,#138531);
#110228=AXIS2_PLACEMENT_3D('',#253454,#138532,#138533);
#110229=AXIS2_PLACEMENT_3D('',#253455,#138534,#138535);
#110230=AXIS2_PLACEMENT_3D('',#253456,#138536,#138537);
#110231=AXIS2_PLACEMENT_3D('',#253459,#138538,#138539);
#110232=AXIS2_PLACEMENT_3D('',#253461,#138540,#138541);
#110233=AXIS2_PLACEMENT_3D('',#253463,#138542,#138543);
#110234=AXIS2_PLACEMENT_3D('',#253464,#138544,#138545);
#110235=AXIS2_PLACEMENT_3D('',#253465,#138546,#138547);
#110236=AXIS2_PLACEMENT_3D('',#253468,#138548,#138549);
#110237=AXIS2_PLACEMENT_3D('',#253470,#138550,#138551);
#110238=AXIS2_PLACEMENT_3D('',#253472,#138552,#138553);
#110239=AXIS2_PLACEMENT_3D('',#253473,#138554,#138555);
#110240=AXIS2_PLACEMENT_3D('',#253485,#138556,#138557);
#110241=AXIS2_PLACEMENT_3D('',#253487,#138558,#138559);
#110242=AXIS2_PLACEMENT_3D('',#253489,#138560,#138561);
#110243=AXIS2_PLACEMENT_3D('',#253490,#138562,#138563);
#110244=AXIS2_PLACEMENT_3D('',#253502,#138564,#138565);
#110245=AXIS2_PLACEMENT_3D('',#253504,#138566,#138567);
#110246=AXIS2_PLACEMENT_3D('',#253506,#138568,#138569);
#110247=AXIS2_PLACEMENT_3D('',#253507,#138570,#138571);
#110248=AXIS2_PLACEMENT_3D('',#253519,#138572,#138573);
#110249=AXIS2_PLACEMENT_3D('',#253521,#138574,#138575);
#110250=AXIS2_PLACEMENT_3D('',#253523,#138576,#138577);
#110251=AXIS2_PLACEMENT_3D('',#253524,#138578,#138579);
#110252=AXIS2_PLACEMENT_3D('',#253525,#138580,#138581);
#110253=AXIS2_PLACEMENT_3D('',#253527,#138582,#138583);
#110254=AXIS2_PLACEMENT_3D('',#253529,#138584,#138585);
#110255=AXIS2_PLACEMENT_3D('',#253530,#138586,#138587);
#110256=AXIS2_PLACEMENT_3D('',#253541,#138588,#138589);
#110257=AXIS2_PLACEMENT_3D('',#253543,#138590,#138591);
#110258=AXIS2_PLACEMENT_3D('',#253544,#138592,#138593);
#110259=AXIS2_PLACEMENT_3D('',#253545,#138594,#138595);
#110260=AXIS2_PLACEMENT_3D('',#253549,#138597,#138598);
#110261=AXIS2_PLACEMENT_3D('',#253579,#138600,#138601);
#110262=AXIS2_PLACEMENT_3D('',#253629,#138603,#138604);
#110263=AXIS2_PLACEMENT_3D('',#253631,#138606,#138607);
#110264=AXIS2_PLACEMENT_3D('',#253634,#138608,#138609);
#110265=AXIS2_PLACEMENT_3D('',#253639,#138610,#138611);
#110266=AXIS2_PLACEMENT_3D('',#253644,#138612,#138613);
#110267=AXIS2_PLACEMENT_3D('',#253646,#138614,#138615);
#110268=AXIS2_PLACEMENT_3D('',#253649,#138617,#138618);
#110269=AXIS2_PLACEMENT_3D('',#253650,#138619,#138620);
#110270=AXIS2_PLACEMENT_3D('',#253652,#138621,#138622);
#110271=AXIS2_PLACEMENT_3D('',#253655,#138624,#138625);
#110272=AXIS2_PLACEMENT_3D('',#253656,#138626,#138627);
#110273=AXIS2_PLACEMENT_3D('',#253658,#138628,#138629);
#110274=AXIS2_PLACEMENT_3D('',#253661,#138631,#138632);
#110275=AXIS2_PLACEMENT_3D('',#253662,#138633,#138634);
#110276=AXIS2_PLACEMENT_3D('',#253664,#138635,#138636);
#110277=AXIS2_PLACEMENT_3D('',#253667,#138638,#138639);
#110278=AXIS2_PLACEMENT_3D('',#253668,#138640,#138641);
#110279=AXIS2_PLACEMENT_3D('',#253670,#138642,#138643);
#110280=AXIS2_PLACEMENT_3D('',#253673,#138645,#138646);
#110281=AXIS2_PLACEMENT_3D('',#253674,#138647,#138648);
#110282=AXIS2_PLACEMENT_3D('',#253678,#138650,#138651);
#110283=AXIS2_PLACEMENT_3D('',#253680,#138653,#138654);
#110284=AXIS2_PLACEMENT_3D('',#253693,#138655,#138656);
#110285=AXIS2_PLACEMENT_3D('',#253756,#138657,#138658);
#110286=AXIS2_PLACEMENT_3D('',#253873,#138659,#138660);
#110287=AXIS2_PLACEMENT_3D('',#253930,#138661,#138662);
#110288=AXIS2_PLACEMENT_3D('',#253993,#138663,#138664);
#110289=AXIS2_PLACEMENT_3D('',#254050,#138665,#138666);
#110290=AXIS2_PLACEMENT_3D('',#254107,#138667,#138668);
#110291=AXIS2_PLACEMENT_3D('',#254164,#138669,#138670);
#110292=AXIS2_PLACEMENT_3D('',#254175,#138671,#138672);
#110293=AXIS2_PLACEMENT_3D('',#254178,#138673,#138674);
#110294=AXIS2_PLACEMENT_3D('',#254182,#138676,#138677);
#110295=AXIS2_PLACEMENT_3D('',#254193,#138679,#138680);
#110296=AXIS2_PLACEMENT_3D('',#254250,#138682,#138683);
#110297=AXIS2_PLACEMENT_3D('',#254252,#138685,#138686);
#110298=AXIS2_PLACEMENT_3D('',#254255,#138687,#138688);
#110299=AXIS2_PLACEMENT_3D('',#254259,#138690,#138691);
#110300=AXIS2_PLACEMENT_3D('',#254322,#138693,#138694);
#110301=AXIS2_PLACEMENT_3D('',#254379,#138696,#138697);
#110302=AXIS2_PLACEMENT_3D('',#254381,#138699,#138700);
#110303=AXIS2_PLACEMENT_3D('',#254387,#138704,#138705);
#110304=AXIS2_PLACEMENT_3D('',#254390,#138708,#138709);
#110305=AXIS2_PLACEMENT_3D('',#254399,#138714,#138715);
#110306=AXIS2_PLACEMENT_3D('',#254405,#138718,#138719);
#110307=AXIS2_PLACEMENT_3D('',#254464,#138720,#138721);
#110308=AXIS2_PLACEMENT_3D('',#254518,#138722,#138723);
#110309=AXIS2_PLACEMENT_3D('',#254519,#138724,#138725);
#110310=AXIS2_PLACEMENT_3D('',#254525,#138728,#138729);
#110311=AXIS2_PLACEMENT_3D('',#254585,#138730,#138731);
#110312=AXIS2_PLACEMENT_3D('',#254595,#138733,#138734);
#110313=AXIS2_PLACEMENT_3D('',#254596,#138735,#138736);
#110314=AXIS2_PLACEMENT_3D('',#254660,#138740,#138741);
#110315=AXIS2_PLACEMENT_3D('',#254665,#138743,#138744);
#110316=AXIS2_PLACEMENT_3D('',#254668,#138746,#138747);
#110317=AXIS2_PLACEMENT_3D('',#254669,#138748,#138749);
#110318=AXIS2_PLACEMENT_3D('',#254675,#138753,#138754);
#110319=AXIS2_PLACEMENT_3D('',#254677,#138755,#138756);
#110320=AXIS2_PLACEMENT_3D('',#254680,#138758,#138759);
#110321=AXIS2_PLACEMENT_3D('',#254681,#138760,#138761);
#110322=AXIS2_PLACEMENT_3D('',#254687,#138765,#138766);
#110323=AXIS2_PLACEMENT_3D('',#254689,#138767,#138768);
#110324=AXIS2_PLACEMENT_3D('',#254692,#138770,#138771);
#110325=AXIS2_PLACEMENT_3D('',#254693,#138772,#138773);
#110326=AXIS2_PLACEMENT_3D('',#254699,#138777,#138778);
#110327=AXIS2_PLACEMENT_3D('',#254701,#138779,#138780);
#110328=AXIS2_PLACEMENT_3D('',#254704,#138782,#138783);
#110329=AXIS2_PLACEMENT_3D('',#254705,#138784,#138785);
#110330=AXIS2_PLACEMENT_3D('',#254708,#138788,#138789);
#110331=AXIS2_PLACEMENT_3D('',#254759,#138791,#138792);
#110332=AXIS2_PLACEMENT_3D('',#254808,#138794,#138795);
#110333=AXIS2_PLACEMENT_3D('',#254847,#138799,#138800);
#110334=AXIS2_PLACEMENT_3D('',#254848,#138801,#138802);
#110335=AXIS2_PLACEMENT_3D('',#254860,#138805,#138806);
#110336=AXIS2_PLACEMENT_3D('',#254888,#138808,#138809);
#110337=AXIS2_PLACEMENT_3D('',#254889,#138810,#138811);
#110338=AXIS2_PLACEMENT_3D('',#254993,#138812,#138813);
#110339=AXIS2_PLACEMENT_3D('',#254996,#138814,#138815);
#110340=AXIS2_PLACEMENT_3D('',#255000,#138817,#138818);
#110341=AXIS2_PLACEMENT_3D('',#255002,#138820,#138821);
#110342=AXIS2_PLACEMENT_3D('',#255022,#138823,#138824);
#110343=AXIS2_PLACEMENT_3D('',#255024,#138825,#138826);
#110344=AXIS2_PLACEMENT_3D('',#255026,#138828,#138829);
#110345=AXIS2_PLACEMENT_3D('',#255029,#138830,#138831);
#110346=AXIS2_PLACEMENT_3D('',#255048,#138834,#138835);
#110347=AXIS2_PLACEMENT_3D('',#255049,#138836,#138837);
#110348=AXIS2_PLACEMENT_3D('',#255050,#138838,#138839);
#110349=AXIS2_PLACEMENT_3D('',#255053,#138840,#138841);
#110350=AXIS2_PLACEMENT_3D('',#255056,#138844,#138845);
#110351=AXIS2_PLACEMENT_3D('',#255061,#138847,#138848);
#110352=AXIS2_PLACEMENT_3D('',#255064,#138850,#138851);
#110353=AXIS2_PLACEMENT_3D('',#255065,#138852,#138853);
#110354=AXIS2_PLACEMENT_3D('',#255066,#138854,#138855);
#110355=AXIS2_PLACEMENT_3D('',#255067,#138856,#138857);
#110356=AXIS2_PLACEMENT_3D('',#255072,#138859,#138860);
#110357=AXIS2_PLACEMENT_3D('',#255075,#138862,#138863);
#110358=AXIS2_PLACEMENT_3D('',#255076,#138864,#138865);
#110359=AXIS2_PLACEMENT_3D('',#255081,#138867,#138868);
#110360=AXIS2_PLACEMENT_3D('',#255084,#138870,#138871);
#110361=AXIS2_PLACEMENT_3D('',#255085,#138872,#138873);
#110362=AXIS2_PLACEMENT_3D('',#255089,#138875,#138876);
#110363=AXIS2_PLACEMENT_3D('',#255091,#138878,#138879);
#110364=AXIS2_PLACEMENT_3D('',#255095,#138881,#138882);
#110365=AXIS2_PLACEMENT_3D('',#255097,#138884,#138885);
#110366=AXIS2_PLACEMENT_3D('',#255162,#138888,#138889);
#110367=AXIS2_PLACEMENT_3D('',#255224,#138892,#138893);
#110368=AXIS2_PLACEMENT_3D('',#255288,#138896,#138897);
#110369=AXIS2_PLACEMENT_3D('',#255291,#138898,#138899);
#110370=AXIS2_PLACEMENT_3D('',#255295,#138901,#138902);
#110371=AXIS2_PLACEMENT_3D('',#255297,#138904,#138905);
#110372=AXIS2_PLACEMENT_3D('',#255299,#138907,#138908);
#110373=AXIS2_PLACEMENT_3D('',#255360,#138911,#138912);
#110374=AXIS2_PLACEMENT_3D('',#255427,#138916,#138917);
#110375=AXIS2_PLACEMENT_3D('',#255430,#138918,#138919);
#110376=AXIS2_PLACEMENT_3D('',#255434,#138921,#138922);
#110377=AXIS2_PLACEMENT_3D('',#255438,#138924,#138925);
#110378=AXIS2_PLACEMENT_3D('',#255440,#138926,#138927);
#110379=AXIS2_PLACEMENT_3D('',#255442,#138928,#138929);
#110380=AXIS2_PLACEMENT_3D('',#255444,#138931,#138932);
#110381=AXIS2_PLACEMENT_3D('',#255508,#138936,#138937);
#110382=AXIS2_PLACEMENT_3D('',#255574,#138941,#138942);
#110383=AXIS2_PLACEMENT_3D('',#255577,#138943,#138944);
#110384=AXIS2_PLACEMENT_3D('',#255581,#138946,#138947);
#110385=AXIS2_PLACEMENT_3D('',#255584,#138950,#138951);
#110386=AXIS2_PLACEMENT_3D('',#255588,#138953,#138954);
#110387=AXIS2_PLACEMENT_3D('',#255591,#138957,#138958);
#110388=AXIS2_PLACEMENT_3D('',#255592,#138959,#138960);
#110389=AXIS2_PLACEMENT_3D('',#255593,#138961,#138962);
#110390=AXIS2_PLACEMENT_3D('',#255594,#138963,#138964);
#110391=AXIS2_PLACEMENT_3D('',#255595,#138965,#138966);
#110392=AXIS2_PLACEMENT_3D('',#255600,#138967,#138968);
#110393=AXIS2_PLACEMENT_3D('',#255601,#138969,#138970);
#110394=AXIS2_PLACEMENT_3D('',#255606,#138971,#138972);
#110395=AXIS2_PLACEMENT_3D('',#255615,#138973,#138974);
#110396=AXIS2_PLACEMENT_3D('',#255624,#138975,#138976);
#110397=AXIS2_PLACEMENT_3D('',#255626,#138977,#138978);
#110398=AXIS2_PLACEMENT_3D('',#255694,#138979,#138980);
#110399=AXIS2_PLACEMENT_3D('',#255719,#138981,#138982);
#110400=AXIS2_PLACEMENT_3D('',#255788,#138983,#138984);
#110401=AXIS2_PLACEMENT_3D('',#255789,#138985,#138986);
#110402=AXIS2_PLACEMENT_3D('',#255814,#138987,#138988);
#110403=AXIS2_PLACEMENT_3D('',#255816,#138989,#138990);
#110404=AXIS2_PLACEMENT_3D('',#255908,#138991,#138992);
#110405=AXIS2_PLACEMENT_3D('',#255941,#138993,#138994);
#110406=AXIS2_PLACEMENT_3D('',#255966,#138995,#138996);
#110407=AXIS2_PLACEMENT_3D('',#255968,#138997,#138998);
#110408=AXIS2_PLACEMENT_3D('',#256060,#138999,#139000);
#110409=AXIS2_PLACEMENT_3D('',#256129,#139001,#139002);
#110410=AXIS2_PLACEMENT_3D('',#256211,#139003,#139004);
#110411=AXIS2_PLACEMENT_3D('',#256212,#139005,#139006);
#110412=AXIS2_PLACEMENT_3D('',#256213,#139007,#139008);
#110413=AXIS2_PLACEMENT_3D('',#256214,#139009,#139010);
#110414=AXIS2_PLACEMENT_3D('',#256215,#139011,#139012);
#110415=AXIS2_PLACEMENT_3D('',#256216,#139013,#139014);
#110416=AXIS2_PLACEMENT_3D('',#256217,#139015,#139016);
#110417=AXIS2_PLACEMENT_3D('',#256218,#139017,#139018);
#110418=AXIS2_PLACEMENT_3D('',#256228,#139019,#139020);
#110419=AXIS2_PLACEMENT_3D('',#256320,#139021,#139022);
#110420=AXIS2_PLACEMENT_3D('',#256321,#139023,#139024);
#110421=AXIS2_PLACEMENT_3D('',#256322,#139025,#139026);
#110422=AXIS2_PLACEMENT_3D('',#256372,#139027,#139028);
#110423=AXIS2_PLACEMENT_3D('',#256373,#139029,#139030);
#110424=AXIS2_PLACEMENT_3D('',#256416,#139031,#139032);
#110425=AXIS2_PLACEMENT_3D('',#256417,#139033,#139034);
#110426=AXIS2_PLACEMENT_3D('',#256418,#139035,#139036);
#110427=AXIS2_PLACEMENT_3D('',#256419,#139037,#139038);
#110428=AXIS2_PLACEMENT_3D('',#256511,#139039,#139040);
#110429=AXIS2_PLACEMENT_3D('',#256512,#139041,#139042);
#110430=AXIS2_PLACEMENT_3D('',#256513,#139043,#139044);
#110431=AXIS2_PLACEMENT_3D('',#256563,#139045,#139046);
#110432=AXIS2_PLACEMENT_3D('',#256564,#139047,#139048);
#110433=AXIS2_PLACEMENT_3D('',#256607,#139049,#139050);
#110434=AXIS2_PLACEMENT_3D('',#256608,#139051,#139052);
#110435=AXIS2_PLACEMENT_3D('',#256609,#139053,#139054);
#110436=AXIS2_PLACEMENT_3D('',#256610,#139055,#139056);
#110437=AXIS2_PLACEMENT_3D('',#256611,#139057,#139058);
#110438=AXIS2_PLACEMENT_3D('',#256703,#139059,#139060);
#110439=AXIS2_PLACEMENT_3D('',#256704,#139061,#139062);
#110440=AXIS2_PLACEMENT_3D('',#256705,#139063,#139064);
#110441=AXIS2_PLACEMENT_3D('',#256755,#139065,#139066);
#110442=AXIS2_PLACEMENT_3D('',#256756,#139067,#139068);
#110443=AXIS2_PLACEMENT_3D('',#256799,#139069,#139070);
#110444=AXIS2_PLACEMENT_3D('',#256800,#139071,#139072);
#110445=AXIS2_PLACEMENT_3D('',#256843,#139073,#139074);
#110446=AXIS2_PLACEMENT_3D('',#256844,#139075,#139076);
#110447=AXIS2_PLACEMENT_3D('',#256845,#139077,#139078);
#110448=AXIS2_PLACEMENT_3D('',#256846,#139079,#139080);
#110449=AXIS2_PLACEMENT_3D('',#256847,#139081,#139082);
#110450=AXIS2_PLACEMENT_3D('',#256948,#139083,#139084);
#110451=AXIS2_PLACEMENT_3D('',#256949,#139085,#139086);
#110452=AXIS2_PLACEMENT_3D('',#256950,#139087,#139088);
#110453=AXIS2_PLACEMENT_3D('',#256951,#139089,#139090);
#110454=AXIS2_PLACEMENT_3D('',#257052,#139091,#139092);
#110455=AXIS2_PLACEMENT_3D('',#257153,#139093,#139094);
#110456=AXIS2_PLACEMENT_3D('',#257245,#139095,#139096);
#110457=AXIS2_PLACEMENT_3D('',#257346,#139097,#139098);
#110458=AXIS2_PLACEMENT_3D('',#257447,#139099,#139100);
#110459=AXIS2_PLACEMENT_3D('',#257548,#139101,#139102);
#110460=AXIS2_PLACEMENT_3D('',#257549,#139103,#139104);
#110461=AXIS2_PLACEMENT_3D('',#257550,#139105,#139106);
#110462=AXIS2_PLACEMENT_3D('',#257551,#139107,#139108);
#110463=AXIS2_PLACEMENT_3D('',#257889,#139109,#139110);
#110464=AXIS2_PLACEMENT_3D('',#257890,#139111,#139112);
#110465=AXIS2_PLACEMENT_3D('',#257891,#139113,#139114);
#110466=AXIS2_PLACEMENT_3D('',#258357,#139115,#139116);
#110467=AXIS2_PLACEMENT_3D('',#258358,#139117,#139118);
#110468=AXIS2_PLACEMENT_3D('',#258359,#139119,#139120);
#110469=AXIS2_PLACEMENT_3D('',#258825,#139121,#139122);
#110470=AXIS2_PLACEMENT_3D('',#258826,#139123,#139124);
#110471=AXIS2_PLACEMENT_3D('',#258827,#139125,#139126);
#110472=AXIS2_PLACEMENT_3D('',#259006,#139127,#139128);
#110473=AXIS2_PLACEMENT_3D('',#259235,#139129,#139130);
#110474=AXIS2_PLACEMENT_3D('',#259236,#139131,#139132);
#110475=AXIS2_PLACEMENT_3D('',#259237,#139133,#139134);
#110476=AXIS2_PLACEMENT_3D('',#259539,#139135,#139136);
#110477=AXIS2_PLACEMENT_3D('',#259552,#139137,#139138);
#110478=AXIS2_PLACEMENT_3D('',#259553,#139139,#139140);
#110479=AXIS2_PLACEMENT_3D('',#259612,#139141,#139142);
#110480=AXIS2_PLACEMENT_3D('',#259625,#139143,#139144);
#110481=AXIS2_PLACEMENT_3D('',#259626,#139145,#139146);
#110482=AXIS2_PLACEMENT_3D('',#259651,#139147,#139148);
#110483=AXIS2_PLACEMENT_3D('',#259652,#139149,#139150);
#110484=AXIS2_PLACEMENT_3D('',#259671,#139151,#139152);
#110485=AXIS2_PLACEMENT_3D('',#259672,#139153,#139154);
#110486=AXIS2_PLACEMENT_3D('',#259737,#139155,#139156);
#110487=AXIS2_PLACEMENT_3D('',#259810,#139157,#139158);
#110488=AXIS2_PLACEMENT_3D('',#259823,#139159,#139160);
#110489=AXIS2_PLACEMENT_3D('',#259944,#139161,#139162);
#110490=AXIS2_PLACEMENT_3D('',#259957,#139163,#139164);
#110491=AXIS2_PLACEMENT_3D('',#260084,#139165,#139166);
#110492=AXIS2_PLACEMENT_3D('',#260097,#139167,#139168);
#110493=AXIS2_PLACEMENT_3D('',#260218,#139169,#139170);
#110494=AXIS2_PLACEMENT_3D('',#260231,#139171,#139172);
#110495=AXIS2_PLACEMENT_3D('',#260358,#139173,#139174);
#110496=AXIS2_PLACEMENT_3D('',#260371,#139175,#139176);
#110497=AXIS2_PLACEMENT_3D('',#260492,#139177,#139178);
#110498=AXIS2_PLACEMENT_3D('',#260505,#139179,#139180);
#110499=AXIS2_PLACEMENT_3D('',#260530,#139181,#139182);
#110500=AXIS2_PLACEMENT_3D('',#260543,#139183,#139184);
#110501=AXIS2_PLACEMENT_3D('',#260766,#139185,#139186);
#110502=AXIS2_PLACEMENT_3D('',#260779,#139187,#139188);
#110503=AXIS2_PLACEMENT_3D('',#260834,#139189,#139190);
#110504=AXIS2_PLACEMENT_3D('',#260835,#139191,#139192);
#110505=AXIS2_PLACEMENT_3D('',#260892,#139193,#139194);
#110506=AXIS2_PLACEMENT_3D('',#260893,#139195,#139196);
#110507=AXIS2_PLACEMENT_3D('',#260908,#139197,#139198);
#110508=AXIS2_PLACEMENT_3D('',#260909,#139199,#139200);
#110509=AXIS2_PLACEMENT_3D('',#260912,#139201,#139202);
#110510=AXIS2_PLACEMENT_3D('',#260913,#139203,#139204);
#110511=AXIS2_PLACEMENT_3D('',#260916,#139205,#139206);
#110512=AXIS2_PLACEMENT_3D('',#260918,#139207,#139208);
#110513=AXIS2_PLACEMENT_3D('',#260919,#139209,#139210);
#110514=AXIS2_PLACEMENT_3D('',#260920,#139211,#139212);
#110515=AXIS2_PLACEMENT_3D('',#260921,#139213,#139214);
#110516=AXIS2_PLACEMENT_3D('',#260924,#139215,#139216);
#110517=AXIS2_PLACEMENT_3D('',#260926,#139217,#139218);
#110518=AXIS2_PLACEMENT_3D('',#260927,#139219,#139220);
#110519=AXIS2_PLACEMENT_3D('',#260928,#139221,#139222);
#110520=AXIS2_PLACEMENT_3D('',#261224,#139223,#139224);
#110521=AXIS2_PLACEMENT_3D('',#261264,#139225,#139226);
#110522=AXIS2_PLACEMENT_3D('',#261266,#139227,#139228);
#110523=AXIS2_PLACEMENT_3D('',#261273,#139229,#139230);
#110524=AXIS2_PLACEMENT_3D('',#261324,#139231,#139232);
#110525=AXIS2_PLACEMENT_3D('',#261326,#139233,#139234);
#110526=AXIS2_PLACEMENT_3D('',#261329,#139236,#139237);
#110527=AXIS2_PLACEMENT_3D('',#261410,#139238,#139239);
#110528=AXIS2_PLACEMENT_3D('',#261412,#139241,#139242);
#110529=AXIS2_PLACEMENT_3D('',#261414,#139243,#139244);
#110530=AXIS2_PLACEMENT_3D('',#261415,#139245,#139246);
#110531=AXIS2_PLACEMENT_3D('',#261476,#139247,#139248);
#110532=AXIS2_PLACEMENT_3D('',#261479,#139249,#139250);
#110533=AXIS2_PLACEMENT_3D('',#261481,#139251,#139252);
#110534=AXIS2_PLACEMENT_3D('',#261482,#139253,#139254);
#110535=AXIS2_PLACEMENT_3D('',#261483,#139255,#139256);
#110536=AXIS2_PLACEMENT_3D('',#261484,#139257,#139258);
#110537=AXIS2_PLACEMENT_3D('',#261486,#139259,#139260);
#110538=AXIS2_PLACEMENT_3D('',#261488,#139261,#139262);
#110539=AXIS2_PLACEMENT_3D('',#261490,#139263,#139264);
#110540=AXIS2_PLACEMENT_3D('',#261491,#139265,#139266);
#110541=AXIS2_PLACEMENT_3D('',#261492,#139267,#139268);
#110542=AXIS2_PLACEMENT_3D('',#261568,#139270,#139271);
#110543=AXIS2_PLACEMENT_3D('',#261570,#139272,#139273);
#110544=AXIS2_PLACEMENT_3D('',#261572,#139275,#139276);
#110545=AXIS2_PLACEMENT_3D('',#261575,#139278,#139279);
#110546=AXIS2_PLACEMENT_3D('',#261576,#139280,#139281);
#110547=AXIS2_PLACEMENT_3D('',#261577,#139282,#139283);
#110548=AXIS2_PLACEMENT_3D('',#261578,#139284,#139285);
#110549=AXIS2_PLACEMENT_3D('',#261580,#139286,#139287);
#110550=AXIS2_PLACEMENT_3D('',#261582,#139288,#139289);
#110551=AXIS2_PLACEMENT_3D('',#261583,#139290,#139291);
#110552=AXIS2_PLACEMENT_3D('',#261584,#139292,#139293);
#110553=AXIS2_PLACEMENT_3D('',#261586,#139294,#139295);
#110554=AXIS2_PLACEMENT_3D('',#261588,#139296,#139297);
#110555=AXIS2_PLACEMENT_3D('',#261590,#139298,#139299);
#110556=AXIS2_PLACEMENT_3D('',#261591,#139300,#139301);
#110557=AXIS2_PLACEMENT_3D('',#261592,#139302,#139303);
#110558=AXIS2_PLACEMENT_3D('',#261595,#139304,#139305);
#110559=AXIS2_PLACEMENT_3D('',#261596,#139306,#139307);
#110560=AXIS2_PLACEMENT_3D('',#261598,#139308,#139309);
#110561=AXIS2_PLACEMENT_3D('',#261599,#139310,#139311);
#110562=AXIS2_PLACEMENT_3D('',#261600,#139312,#139313);
#110563=AXIS2_PLACEMENT_3D('',#261602,#139314,#139315);
#110564=AXIS2_PLACEMENT_3D('',#261604,#139316,#139317);
#110565=AXIS2_PLACEMENT_3D('',#261605,#139318,#139319);
#110566=AXIS2_PLACEMENT_3D('',#261606,#139320,#139321);
#110567=AXIS2_PLACEMENT_3D('',#261608,#139322,#139323);
#110568=AXIS2_PLACEMENT_3D('',#261610,#139324,#139325);
#110569=AXIS2_PLACEMENT_3D('',#261611,#139326,#139327);
#110570=AXIS2_PLACEMENT_3D('',#261612,#139328,#139329);
#110571=AXIS2_PLACEMENT_3D('',#261614,#139330,#139331);
#110572=AXIS2_PLACEMENT_3D('',#261617,#139333,#139334);
#110573=AXIS2_PLACEMENT_3D('',#261618,#139335,#139336);
#110574=AXIS2_PLACEMENT_3D('',#261620,#139338,#139339);
#110575=AXIS2_PLACEMENT_3D('',#261622,#139341,#139342);
#110576=AXIS2_PLACEMENT_3D('',#261624,#139343,#139344);
#110577=AXIS2_PLACEMENT_3D('',#261626,#139346,#139347);
#110578=AXIS2_PLACEMENT_3D('',#261629,#139349,#139350);
#110579=AXIS2_PLACEMENT_3D('',#261630,#139351,#139352);
#110580=AXIS2_PLACEMENT_3D('',#261632,#139353,#139354);
#110581=AXIS2_PLACEMENT_3D('',#261635,#139356,#139357);
#110582=AXIS2_PLACEMENT_3D('',#261636,#139358,#139359);
#110583=AXIS2_PLACEMENT_3D('',#261637,#139360,#139361);
#110584=AXIS2_PLACEMENT_3D('',#261638,#139362,#139363);
#110585=AXIS2_PLACEMENT_3D('',#261639,#139364,#139365);
#110586=AXIS2_PLACEMENT_3D('',#261640,#139366,#139367);
#110587=AXIS2_PLACEMENT_3D('',#261641,#139368,#139369);
#110588=AXIS2_PLACEMENT_3D('',#261662,#139371,#139372);
#110589=AXIS2_PLACEMENT_3D('',#261678,#139373,#139374);
#110590=AXIS2_PLACEMENT_3D('',#261716,#139376,#139377);
#110591=AXIS2_PLACEMENT_3D('',#261754,#139379,#139380);
#110592=AXIS2_PLACEMENT_3D('',#261792,#139382,#139383);
#110593=AXIS2_PLACEMENT_3D('',#261830,#139385,#139386);
#110594=AXIS2_PLACEMENT_3D('',#261868,#139388,#139389);
#110595=AXIS2_PLACEMENT_3D('',#261883,#139391,#139392);
#110596=AXIS2_PLACEMENT_3D('',#261884,#139393,#139394);
#110597=AXIS2_PLACEMENT_3D('',#261925,#139396,#139397);
#110598=AXIS2_PLACEMENT_3D('',#261938,#139398,#139399);
#110599=AXIS2_PLACEMENT_3D('',#262014,#139401,#139402);
#110600=AXIS2_PLACEMENT_3D('',#262090,#139404,#139405);
#110601=AXIS2_PLACEMENT_3D('',#262166,#139407,#139408);
#110602=AXIS2_PLACEMENT_3D('',#262242,#139410,#139411);
#110603=AXIS2_PLACEMENT_3D('',#262320,#139413,#139414);
#110604=AXIS2_PLACEMENT_3D('',#262325,#139416,#139417);
#110605=AXIS2_PLACEMENT_3D('',#262386,#139418,#139419);
#110606=AXIS2_PLACEMENT_3D('',#262388,#139420,#139421);
#110607=AXIS2_PLACEMENT_3D('',#262390,#139422,#139423);
#110608=AXIS2_PLACEMENT_3D('',#262391,#139424,#139425);
#110609=AXIS2_PLACEMENT_3D('',#262394,#139427,#139428);
#110610=AXIS2_PLACEMENT_3D('',#262395,#139429,#139430);
#110611=AXIS2_PLACEMENT_3D('',#262398,#139431,#139432);
#110612=AXIS2_PLACEMENT_3D('',#262399,#139433,#139434);
#110613=AXIS2_PLACEMENT_3D('',#262400,#139435,#139436);
#110614=AXIS2_PLACEMENT_3D('',#262401,#139437,#139438);
#110615=AXIS2_PLACEMENT_3D('',#262404,#139440,#139441);
#110616=AXIS2_PLACEMENT_3D('',#262405,#139442,#139443);
#110617=AXIS2_PLACEMENT_3D('',#262426,#139444,#139445);
#110618=AXIS2_PLACEMENT_3D('',#262427,#139446,#139447);
#110619=AXIS2_PLACEMENT_3D('',#262430,#139448,#139449);
#110620=AXIS2_PLACEMENT_3D('',#262432,#139450,#139451);
#110621=AXIS2_PLACEMENT_3D('',#262434,#139452,#139453);
#110622=AXIS2_PLACEMENT_3D('',#262436,#139454,#139455);
#110623=AXIS2_PLACEMENT_3D('',#262438,#139456,#139457);
#110624=AXIS2_PLACEMENT_3D('',#262439,#139458,#139459);
#110625=AXIS2_PLACEMENT_3D('',#262440,#139460,#139461);
#110626=AXIS2_PLACEMENT_3D('',#262444,#139462,#139463);
#110627=AXIS2_PLACEMENT_3D('',#262448,#139464,#139465);
#110628=AXIS2_PLACEMENT_3D('',#262452,#139466,#139467);
#110629=AXIS2_PLACEMENT_3D('',#262456,#139468,#139469);
#110630=AXIS2_PLACEMENT_3D('',#262460,#139470,#139471);
#110631=AXIS2_PLACEMENT_3D('',#262464,#139472,#139473);
#110632=AXIS2_PLACEMENT_3D('',#262477,#139480,#139481);
#110633=AXIS2_PLACEMENT_3D('',#262480,#139484,#139485);
#110634=AXIS2_PLACEMENT_3D('',#262482,#139487,#139488);
#110635=AXIS2_PLACEMENT_3D('',#262484,#139490,#139491);
#110636=AXIS2_PLACEMENT_3D('',#262486,#139493,#139494);
#110637=AXIS2_PLACEMENT_3D('',#262488,#139496,#139497);
#110638=AXIS2_PLACEMENT_3D('',#262828,#139498,#139499);
#110639=AXIS2_PLACEMENT_3D('',#263168,#139500,#139501);
#110640=AXIS2_PLACEMENT_3D('',#263189,#139503,#139504);
#110641=AXIS2_PLACEMENT_3D('',#263205,#139505,#139506);
#110642=AXIS2_PLACEMENT_3D('',#263243,#139508,#139509);
#110643=AXIS2_PLACEMENT_3D('',#263281,#139511,#139512);
#110644=AXIS2_PLACEMENT_3D('',#263319,#139514,#139515);
#110645=AXIS2_PLACEMENT_3D('',#263357,#139517,#139518);
#110646=AXIS2_PLACEMENT_3D('',#263395,#139520,#139521);
#110647=AXIS2_PLACEMENT_3D('',#263410,#139523,#139524);
#110648=AXIS2_PLACEMENT_3D('',#263411,#139525,#139526);
#110649=AXIS2_PLACEMENT_3D('',#263452,#139528,#139529);
#110650=AXIS2_PLACEMENT_3D('',#263465,#139530,#139531);
#110651=AXIS2_PLACEMENT_3D('',#263541,#139533,#139534);
#110652=AXIS2_PLACEMENT_3D('',#263617,#139536,#139537);
#110653=AXIS2_PLACEMENT_3D('',#263693,#139539,#139540);
#110654=AXIS2_PLACEMENT_3D('',#263769,#139542,#139543);
#110655=AXIS2_PLACEMENT_3D('',#263847,#139545,#139546);
#110656=AXIS2_PLACEMENT_3D('',#263852,#139548,#139549);
#110657=AXIS2_PLACEMENT_3D('',#263913,#139550,#139551);
#110658=AXIS2_PLACEMENT_3D('',#263915,#139552,#139553);
#110659=AXIS2_PLACEMENT_3D('',#263917,#139554,#139555);
#110660=AXIS2_PLACEMENT_3D('',#263918,#139556,#139557);
#110661=AXIS2_PLACEMENT_3D('',#263921,#139559,#139560);
#110662=AXIS2_PLACEMENT_3D('',#263922,#139561,#139562);
#110663=AXIS2_PLACEMENT_3D('',#263925,#139563,#139564);
#110664=AXIS2_PLACEMENT_3D('',#263926,#139565,#139566);
#110665=AXIS2_PLACEMENT_3D('',#263927,#139567,#139568);
#110666=AXIS2_PLACEMENT_3D('',#263928,#139569,#139570);
#110667=AXIS2_PLACEMENT_3D('',#263931,#139572,#139573);
#110668=AXIS2_PLACEMENT_3D('',#263932,#139574,#139575);
#110669=AXIS2_PLACEMENT_3D('',#263953,#139576,#139577);
#110670=AXIS2_PLACEMENT_3D('',#263954,#139578,#139579);
#110671=AXIS2_PLACEMENT_3D('',#263957,#139580,#139581);
#110672=AXIS2_PLACEMENT_3D('',#263959,#139582,#139583);
#110673=AXIS2_PLACEMENT_3D('',#263961,#139584,#139585);
#110674=AXIS2_PLACEMENT_3D('',#263963,#139586,#139587);
#110675=AXIS2_PLACEMENT_3D('',#263965,#139588,#139589);
#110676=AXIS2_PLACEMENT_3D('',#263966,#139590,#139591);
#110677=AXIS2_PLACEMENT_3D('',#263967,#139592,#139593);
#110678=AXIS2_PLACEMENT_3D('',#263971,#139594,#139595);
#110679=AXIS2_PLACEMENT_3D('',#263975,#139596,#139597);
#110680=AXIS2_PLACEMENT_3D('',#263979,#139598,#139599);
#110681=AXIS2_PLACEMENT_3D('',#263983,#139600,#139601);
#110682=AXIS2_PLACEMENT_3D('',#263987,#139602,#139603);
#110683=AXIS2_PLACEMENT_3D('',#263991,#139604,#139605);
#110684=AXIS2_PLACEMENT_3D('',#264004,#139612,#139613);
#110685=AXIS2_PLACEMENT_3D('',#264007,#139616,#139617);
#110686=AXIS2_PLACEMENT_3D('',#264009,#139619,#139620);
#110687=AXIS2_PLACEMENT_3D('',#264011,#139622,#139623);
#110688=AXIS2_PLACEMENT_3D('',#264013,#139625,#139626);
#110689=AXIS2_PLACEMENT_3D('',#264015,#139628,#139629);
#110690=AXIS2_PLACEMENT_3D('',#264355,#139630,#139631);
#110691=AXIS2_PLACEMENT_3D('',#264695,#139632,#139633);
#110692=AXIS2_PLACEMENT_3D('',#264697,#139634,#139635);
#110693=AXIS2_PLACEMENT_3D('',#264700,#139637,#139638);
#110694=AXIS2_PLACEMENT_3D('',#264701,#139639,#139640);
#110695=AXIS2_PLACEMENT_3D('',#264704,#139641,#139642);
#110696=AXIS2_PLACEMENT_3D('',#264705,#139643,#139644);
#110697=AXIS2_PLACEMENT_3D('',#264708,#139646,#139647);
#110698=AXIS2_PLACEMENT_3D('',#264709,#139648,#139649);
#110699=AXIS2_PLACEMENT_3D('',#264711,#139650,#139651);
#110700=AXIS2_PLACEMENT_3D('',#264714,#139653,#139654);
#110701=AXIS2_PLACEMENT_3D('',#264715,#139655,#139656);
#110702=AXIS2_PLACEMENT_3D('',#264718,#139657,#139658);
#110703=AXIS2_PLACEMENT_3D('',#264719,#139659,#139660);
#110704=AXIS2_PLACEMENT_3D('',#264722,#139662,#139663);
#110705=AXIS2_PLACEMENT_3D('',#264723,#139664,#139665);
#110706=AXIS2_PLACEMENT_3D('',#264804,#139668,#139669);
#110707=AXIS2_PLACEMENT_3D('',#264841,#139671,#139672);
#110708=AXIS2_PLACEMENT_3D('',#264882,#139674,#139675);
#110709=AXIS2_PLACEMENT_3D('',#264885,#139678,#139679);
#110710=AXIS2_PLACEMENT_3D('',#264886,#139680,#139681);
#110711=AXIS2_PLACEMENT_3D('',#264887,#139682,#139683);
#110712=AXIS2_PLACEMENT_3D('',#264889,#139684,#139685);
#110713=AXIS2_PLACEMENT_3D('',#264892,#139687,#139688);
#110714=AXIS2_PLACEMENT_3D('',#264893,#139689,#139690);
#110715=AXIS2_PLACEMENT_3D('',#264895,#139691,#139692);
#110716=AXIS2_PLACEMENT_3D('',#264898,#139694,#139695);
#110717=AXIS2_PLACEMENT_3D('',#264899,#139696,#139697);
#110718=AXIS2_PLACEMENT_3D('',#264901,#139698,#139699);
#110719=AXIS2_PLACEMENT_3D('',#264903,#139700,#139701);
#110720=AXIS2_PLACEMENT_3D('',#264905,#139702,#139703);
#110721=AXIS2_PLACEMENT_3D('',#264906,#139704,#139705);
#110722=AXIS2_PLACEMENT_3D('',#264907,#139706,#139707);
#110723=AXIS2_PLACEMENT_3D('',#264909,#139708,#139709);
#110724=AXIS2_PLACEMENT_3D('',#264911,#139711,#139712);
#110725=AXIS2_PLACEMENT_3D('',#264914,#139713,#139714);
#110726=AXIS2_PLACEMENT_3D('',#264918,#139716,#139717);
#110727=AXIS2_PLACEMENT_3D('',#264920,#139719,#139720);
#110728=AXIS2_PLACEMENT_3D('',#264922,#139721,#139722);
#110729=AXIS2_PLACEMENT_3D('',#264925,#139724,#139725);
#110730=AXIS2_PLACEMENT_3D('',#264926,#139726,#139727);
#110731=AXIS2_PLACEMENT_3D('',#264928,#139728,#139729);
#110732=AXIS2_PLACEMENT_3D('',#264931,#139731,#139732);
#110733=AXIS2_PLACEMENT_3D('',#264932,#139733,#139734);
#110734=AXIS2_PLACEMENT_3D('',#264934,#139735,#139736);
#110735=AXIS2_PLACEMENT_3D('',#264937,#139738,#139739);
#110736=AXIS2_PLACEMENT_3D('',#264938,#139740,#139741);
#110737=AXIS2_PLACEMENT_3D('',#264940,#139742,#139743);
#110738=AXIS2_PLACEMENT_3D('',#264943,#139745,#139746);
#110739=AXIS2_PLACEMENT_3D('',#264944,#139747,#139748);
#110740=AXIS2_PLACEMENT_3D('',#264946,#139749,#139750);
#110741=AXIS2_PLACEMENT_3D('',#264949,#139752,#139753);
#110742=AXIS2_PLACEMENT_3D('',#264950,#139754,#139755);
#110743=AXIS2_PLACEMENT_3D('',#264952,#139756,#139757);
#110744=AXIS2_PLACEMENT_3D('',#264955,#139759,#139760);
#110745=AXIS2_PLACEMENT_3D('',#264956,#139761,#139762);
#110746=AXIS2_PLACEMENT_3D('',#264958,#139763,#139764);
#110747=AXIS2_PLACEMENT_3D('',#264961,#139766,#139767);
#110748=AXIS2_PLACEMENT_3D('',#264962,#139768,#139769);
#110749=AXIS2_PLACEMENT_3D('',#264964,#139770,#139771);
#110750=AXIS2_PLACEMENT_3D('',#264967,#139773,#139774);
#110751=AXIS2_PLACEMENT_3D('',#264968,#139775,#139776);
#110752=AXIS2_PLACEMENT_3D('',#264970,#139777,#139778);
#110753=AXIS2_PLACEMENT_3D('',#264973,#139780,#139781);
#110754=AXIS2_PLACEMENT_3D('',#264974,#139782,#139783);
#110755=AXIS2_PLACEMENT_3D('',#264976,#139784,#139785);
#110756=AXIS2_PLACEMENT_3D('',#264979,#139787,#139788);
#110757=AXIS2_PLACEMENT_3D('',#264980,#139789,#139790);
#110758=AXIS2_PLACEMENT_3D('',#264985,#139792,#139793);
#110759=AXIS2_PLACEMENT_3D('',#264988,#139795,#139796);
#110760=AXIS2_PLACEMENT_3D('',#264989,#139797,#139798);
#110761=AXIS2_PLACEMENT_3D('',#264995,#139802,#139803);
#110762=AXIS2_PLACEMENT_3D('',#264997,#139804,#139805);
#110763=AXIS2_PLACEMENT_3D('',#265000,#139807,#139808);
#110764=AXIS2_PLACEMENT_3D('',#265001,#139809,#139810);
#110765=AXIS2_PLACEMENT_3D('',#265007,#139814,#139815);
#110766=AXIS2_PLACEMENT_3D('',#265009,#139816,#139817);
#110767=AXIS2_PLACEMENT_3D('',#265012,#139819,#139820);
#110768=AXIS2_PLACEMENT_3D('',#265013,#139821,#139822);
#110769=AXIS2_PLACEMENT_3D('',#265019,#139826,#139827);
#110770=AXIS2_PLACEMENT_3D('',#265021,#139828,#139829);
#110771=AXIS2_PLACEMENT_3D('',#265024,#139831,#139832);
#110772=AXIS2_PLACEMENT_3D('',#265025,#139833,#139834);
#110773=AXIS2_PLACEMENT_3D('',#265028,#139837,#139838);
#110774=AXIS2_PLACEMENT_3D('',#265033,#139840,#139841);
#110775=AXIS2_PLACEMENT_3D('',#265037,#139843,#139844);
#110776=AXIS2_PLACEMENT_3D('',#265041,#139846,#139847);
#110777=AXIS2_PLACEMENT_3D('',#265044,#139849,#139850);
#110778=AXIS2_PLACEMENT_3D('',#265045,#139851,#139852);
#110779=AXIS2_PLACEMENT_3D('',#265046,#139853,#139854);
#110780=AXIS2_PLACEMENT_3D('',#265047,#139855,#139856);
#110781=AXIS2_PLACEMENT_3D('',#265048,#139857,#139858);
#110782=AXIS2_PLACEMENT_3D('',#265049,#139859,#139860);
#110783=AXIS2_PLACEMENT_3D('',#265052,#139861,#139862);
#110784=AXIS2_PLACEMENT_3D('',#265056,#139864,#139865);
#110785=AXIS2_PLACEMENT_3D('',#265060,#139867,#139868);
#110786=AXIS2_PLACEMENT_3D('',#265064,#139870,#139871);
#110787=AXIS2_PLACEMENT_3D('',#265066,#139873,#139874);
#110788=AXIS2_PLACEMENT_3D('',#265070,#139876,#139877);
#110789=AXIS2_PLACEMENT_3D('',#265072,#139879,#139880);
#110790=AXIS2_PLACEMENT_3D('',#265076,#139883,#139884);
#110791=AXIS2_PLACEMENT_3D('',#265079,#139886,#139887);
#110792=AXIS2_PLACEMENT_3D('',#265080,#139888,#139889);
#110793=AXIS2_PLACEMENT_3D('',#265084,#139892,#139893);
#110794=AXIS2_PLACEMENT_3D('',#265087,#139895,#139896);
#110795=AXIS2_PLACEMENT_3D('',#265088,#139897,#139898);
#110796=AXIS2_PLACEMENT_3D('',#265092,#139901,#139902);
#110797=AXIS2_PLACEMENT_3D('',#265095,#139904,#139905);
#110798=AXIS2_PLACEMENT_3D('',#265096,#139906,#139907);
#110799=AXIS2_PLACEMENT_3D('',#265098,#139909,#139910);
#110800=AXIS2_PLACEMENT_3D('',#265099,#139911,#139912);
#110801=AXIS2_PLACEMENT_3D('',#265100,#139913,#139914);
#110802=AXIS2_PLACEMENT_3D('',#265101,#139915,#139916);
#110803=AXIS2_PLACEMENT_3D('',#265102,#139917,#139918);
#110804=AXIS2_PLACEMENT_3D('',#265103,#139919,#139920);
#110805=AXIS2_PLACEMENT_3D('',#265104,#139921,#139922);
#110806=AXIS2_PLACEMENT_3D('',#265105,#139923,#139924);
#110807=AXIS2_PLACEMENT_3D('',#265106,#139925,#139926);
#110808=AXIS2_PLACEMENT_3D('',#265107,#139927,#139928);
#110809=AXIS2_PLACEMENT_3D('',#265108,#139929,#139930);
#110810=AXIS2_PLACEMENT_3D('',#265109,#139931,#139932);
#110811=AXIS2_PLACEMENT_3D('',#265110,#139933,#139934);
#110812=AXIS2_PLACEMENT_3D('',#265111,#139935,#139936);
#110813=AXIS2_PLACEMENT_3D('',#265112,#139937,#139938);
#110814=AXIS2_PLACEMENT_3D('',#265113,#139939,#139940);
#110815=AXIS2_PLACEMENT_3D('',#265114,#139941,#139942);
#110816=AXIS2_PLACEMENT_3D('',#265115,#139943,#139944);
#110817=AXIS2_PLACEMENT_3D('',#265120,#139946,#139947);
#110818=AXIS2_PLACEMENT_3D('',#265123,#139949,#139950);
#110819=AXIS2_PLACEMENT_3D('',#265124,#139951,#139952);
#110820=AXIS2_PLACEMENT_3D('',#265128,#139954,#139955);
#110821=AXIS2_PLACEMENT_3D('',#265133,#139958,#139959);
#110822=AXIS2_PLACEMENT_3D('',#265135,#139961,#139962);
#110823=AXIS2_PLACEMENT_3D('',#265136,#139963,#139964);
#110824=AXIS2_PLACEMENT_3D('',#265137,#139965,#139966);
#110825=AXIS2_PLACEMENT_3D('',#265138,#139967,#139968);
#110826=AXIS2_PLACEMENT_3D('',#265142,#139970,#139971);
#110827=AXIS2_PLACEMENT_3D('',#265144,#139973,#139974);
#110828=AXIS2_PLACEMENT_3D('',#265146,#139976,#139977);
#110829=AXIS2_PLACEMENT_3D('',#265148,#139979,#139980);
#110830=AXIS2_PLACEMENT_3D('',#265152,#139982,#139983);
#110831=AXIS2_PLACEMENT_3D('',#265154,#139985,#139986);
#110832=AXIS2_PLACEMENT_3D('',#265157,#139989,#139990);
#110833=AXIS2_PLACEMENT_3D('',#265158,#139991,#139992);
#112067=DIRECTION('axis',(0.,0.,1.));
#112068=DIRECTION('refdir',(1.,0.,0.));
#112069=DIRECTION('center_axis',(0.,1.,0.));
#112070=DIRECTION('ref_axis',(0.,0.,1.));
#112071=DIRECTION('center_axis',(0.,1.,0.));
#112072=DIRECTION('ref_axis',(0.,0.,1.));
#112073=DIRECTION('center_axis',(1.,0.,-1.22464679914735E-16));
#112074=DIRECTION('ref_axis',(-1.22464679914735E-16,0.,-1.));
#112075=DIRECTION('center_axis',(0.,1.,0.));
#112076=DIRECTION('ref_axis',(0.,0.,1.));
#112077=DIRECTION('center_axis',(0.,1.,0.));
#112078=DIRECTION('ref_axis',(0.,0.,1.));
#112079=DIRECTION('center_axis',(0.,-1.,0.));
#112080=DIRECTION('ref_axis',(0.,0.,-1.));
#112081=DIRECTION('',(0.,1.,0.));
#112082=DIRECTION('',(0.,-1.,0.));
#112083=DIRECTION('center_axis',(0.,1.,0.));
#112084=DIRECTION('ref_axis',(0.,0.,-1.));
#112085=DIRECTION('center_axis',(0.,-1.,0.));
#112086=DIRECTION('ref_axis',(0.,0.,-1.));
#112087=DIRECTION('center_axis',(0.,1.,0.));
#112088=DIRECTION('ref_axis',(0.,0.,1.));
#112089=DIRECTION('center_axis',(0.,1.,0.));
#112090=DIRECTION('ref_axis',(0.,0.,1.));
#112091=DIRECTION('',(0.,-1.,0.));
#112092=DIRECTION('center_axis',(0.,1.,0.));
#112093=DIRECTION('ref_axis',(0.,0.,1.));
#112094=DIRECTION('center_axis',(0.,-1.,0.));
#112095=DIRECTION('ref_axis',(0.,0.,1.));
#112096=DIRECTION('center_axis',(0.,1.,0.));
#112097=DIRECTION('ref_axis',(0.,0.,1.));
#112098=DIRECTION('center_axis',(0.,1.,0.));
#112099=DIRECTION('ref_axis',(0.,0.,1.));
#112100=DIRECTION('center_axis',(0.,-1.,0.));
#112101=DIRECTION('ref_axis',(0.,0.,-1.));
#112102=DIRECTION('center_axis',(0.,1.,0.));
#112103=DIRECTION('ref_axis',(0.,0.,1.));
#112104=DIRECTION('center_axis',(0.,1.,0.));
#112105=DIRECTION('ref_axis',(0.,0.,1.));
#112106=DIRECTION('center_axis',(0.,1.,0.));
#112107=DIRECTION('ref_axis',(0.,0.,1.));
#112108=DIRECTION('',(1.1501184830626E-16,0.343526423752935,-0.939143011571464));
#112109=DIRECTION('center_axis',(0.,1.,0.));
#112110=DIRECTION('ref_axis',(0.,0.,1.));
#112111=DIRECTION('center_axis',(0.,1.,0.));
#112112=DIRECTION('ref_axis',(0.,0.,1.));
#112113=DIRECTION('center_axis',(-1.,0.,7.36451384826826E-15));
#112114=DIRECTION('ref_axis',(-6.98296267768626E-15,0.,-1.));
#112115=DIRECTION('center_axis',(0.,1.,0.));
#112116=DIRECTION('ref_axis',(0.,0.,1.));
#112117=DIRECTION('center_axis',(0.,1.,0.));
#112118=DIRECTION('ref_axis',(0.,0.,1.));
#112119=DIRECTION('center_axis',(0.,1.,0.));
#112120=DIRECTION('ref_axis',(0.,0.,1.));
#112121=DIRECTION('center_axis',(0.,1.,0.));
#112122=DIRECTION('ref_axis',(0.,0.,1.));
#112123=DIRECTION('center_axis',(-1.,0.,1.22464679914735E-16));
#112124=DIRECTION('ref_axis',(-1.22464679914735E-16,0.,-1.));
#112125=DIRECTION('center_axis',(0.,-1.,0.));
#112126=DIRECTION('ref_axis',(0.,0.,-1.));
#112127=DIRECTION('',(4.24471087982595E-17,0.938010460718684,-0.34660694681775));
#112128=DIRECTION('center_axis',(0.,1.,0.));
#112129=DIRECTION('ref_axis',(0.,0.,1.));
#112130=DIRECTION('center_axis',(0.,1.,0.));
#112131=DIRECTION('ref_axis',(0.,0.,1.));
#112132=DIRECTION('center_axis',(0.,1.,0.));
#112133=DIRECTION('ref_axis',(0.,0.,1.));
#112134=DIRECTION('center_axis',(0.,1.,0.));
#112135=DIRECTION('ref_axis',(0.,0.,1.));
#112136=DIRECTION('center_axis',(-1.,0.,1.22464679914735E-16));
#112137=DIRECTION('ref_axis',(-1.22464679914735E-16,0.,-1.));
#112138=DIRECTION('center_axis',(0.,1.,0.));
#112139=DIRECTION('ref_axis',(0.,0.,1.));
#112140=DIRECTION('center_axis',(0.,1.,0.));
#112141=DIRECTION('ref_axis',(0.,0.,1.));
#112142=DIRECTION('',(0.,1.,0.));
#112143=DIRECTION('center_axis',(0.,1.,0.));
#112144=DIRECTION('ref_axis',(0.,0.,1.));
#112145=DIRECTION('center_axis',(0.,1.,0.));
#112146=DIRECTION('ref_axis',(0.,0.,1.));
#112147=DIRECTION('center_axis',(0.,1.,0.));
#112148=DIRECTION('ref_axis',(0.,0.,1.));
#112149=DIRECTION('center_axis',(0.,-1.,0.));
#112150=DIRECTION('ref_axis',(-1.65389215948552E-15,0.,-1.));
#112151=DIRECTION('center_axis',(0.,-1.,0.));
#112152=DIRECTION('ref_axis',(0.,0.,1.));
#112153=DIRECTION('center_axis',(0.,-1.,0.));
#112154=DIRECTION('ref_axis',(0.,0.,1.));
#112155=DIRECTION('center_axis',(0.,-1.,0.));
#112156=DIRECTION('ref_axis',(0.,0.,1.));
#112157=DIRECTION('center_axis',(0.,-1.,0.));
#112158=DIRECTION('ref_axis',(0.,0.,1.));
#112159=DIRECTION('center_axis',(0.,-1.,0.));
#112160=DIRECTION('ref_axis',(0.,0.,-1.));
#112161=DIRECTION('center_axis',(0.,-1.,0.));
#112162=DIRECTION('ref_axis',(0.,0.,-1.));
#112163=DIRECTION('center_axis',(0.,-1.,0.));
#112164=DIRECTION('ref_axis',(0.,0.,-1.));
#112165=DIRECTION('center_axis',(0.,-1.,0.));
#112166=DIRECTION('ref_axis',(0.,0.,-1.));
#112167=DIRECTION('center_axis',(0.,-1.,0.));
#112168=DIRECTION('ref_axis',(0.,0.,-1.));
#112169=DIRECTION('center_axis',(0.,-1.,0.));
#112170=DIRECTION('ref_axis',(0.,0.,-1.));
#112171=DIRECTION('center_axis',(0.,-1.,0.));
#112172=DIRECTION('ref_axis',(0.,0.,-1.));
#112173=DIRECTION('center_axis',(0.,1.,0.));
#112174=DIRECTION('ref_axis',(0.,0.,-1.));
#112175=DIRECTION('center_axis',(0.,1.,0.));
#112176=DIRECTION('ref_axis',(0.,0.,-1.));
#112177=DIRECTION('center_axis',(0.,1.,0.));
#112178=DIRECTION('ref_axis',(1.01064309961486E-15,0.,1.));
#112179=DIRECTION('center_axis',(0.,1.,0.));
#112180=DIRECTION('ref_axis',(0.,0.,-1.));
#112181=DIRECTION('center_axis',(0.,1.,0.));
#112182=DIRECTION('ref_axis',(0.,0.,-1.));
#112183=DIRECTION('center_axis',(0.5,0.,-0.866025403784439));
#112184=DIRECTION('ref_axis',(-0.866025403784439,0.,-0.5));
#112185=DIRECTION('',(0.,-1.,0.));
#112186=DIRECTION('center_axis',(1.,0.,0.));
#112187=DIRECTION('ref_axis',(0.,0.,-1.));
#112188=DIRECTION('',(0.,1.,0.));
#112189=DIRECTION('',(0.,-1.,0.));
#112190=DIRECTION('center_axis',(0.5,0.,0.866025403784439));
#112191=DIRECTION('ref_axis',(0.866025403784439,0.,-0.5));
#112192=DIRECTION('',(0.,1.,0.));
#112193=DIRECTION('',(0.,-1.,0.));
#112194=DIRECTION('center_axis',(-0.499999999999999,0.,0.866025403784439));
#112195=DIRECTION('ref_axis',(0.866025403784439,0.,0.499999999999999));
#112196=DIRECTION('',(0.,-1.,0.));
#112197=DIRECTION('',(0.,1.,0.));
#112198=DIRECTION('center_axis',(-1.,0.,0.));
#112199=DIRECTION('ref_axis',(0.,0.,1.));
#112200=DIRECTION('',(0.,-1.,0.));
#112201=DIRECTION('',(0.,1.,0.));
#112202=DIRECTION('center_axis',(-0.5,0.,-0.866025403784439));
#112203=DIRECTION('ref_axis',(-0.866025403784439,0.,0.5));
#112204=DIRECTION('',(0.,1.,0.));
#112205=DIRECTION('center_axis',(0.,-1.,0.));
#112206=DIRECTION('ref_axis',(0.,0.,-1.));
#112207=DIRECTION('center_axis',(0.,-1.,0.));
#112208=DIRECTION('ref_axis',(0.,0.,-1.));
#112209=DIRECTION('center_axis',(0.,-1.,0.));
#112210=DIRECTION('ref_axis',(0.,0.,-1.));
#112211=DIRECTION('center_axis',(0.,-1.,0.));
#112212=DIRECTION('ref_axis',(0.,0.,-1.));
#112213=DIRECTION('center_axis',(0.,-1.,0.));
#112214=DIRECTION('ref_axis',(1.89882151931499E-15,0.,1.));
#112215=DIRECTION('center_axis',(0.,0.,-1.));
#112216=DIRECTION('ref_axis',(-1.,0.,0.));
#112217=DIRECTION('center_axis',(0.,0.,1.));
#112218=DIRECTION('ref_axis',(1.,0.,0.));
#112219=DIRECTION('',(0.,0.,-1.));
#112220=DIRECTION('center_axis',(0.,0.,1.));
#112221=DIRECTION('ref_axis',(1.,0.,0.));
#112222=DIRECTION('center_axis',(0.,0.,-1.));
#112223=DIRECTION('ref_axis',(-1.,0.,0.));
#112224=DIRECTION('center_axis',(0.,0.,1.));
#112225=DIRECTION('ref_axis',(1.,0.,0.));
#112226=DIRECTION('',(0.,0.,1.));
#112227=DIRECTION('center_axis',(0.,0.,1.));
#112228=DIRECTION('ref_axis',(1.,0.,0.));
#112229=DIRECTION('center_axis',(0.,0.,1.));
#112230=DIRECTION('ref_axis',(1.,0.,0.));
#112231=DIRECTION('center_axis',(0.,0.,1.));
#112232=DIRECTION('ref_axis',(1.,0.,0.));
#112233=DIRECTION('center_axis',(0.,0.,-1.));
#112234=DIRECTION('ref_axis',(-1.,0.,0.));
#112235=DIRECTION('center_axis',(0.,0.,1.));
#112236=DIRECTION('ref_axis',(1.,0.,0.));
#112237=DIRECTION('',(0.,0.,-1.));
#112238=DIRECTION('center_axis',(0.,0.,1.));
#112239=DIRECTION('ref_axis',(1.,0.,0.));
#112240=DIRECTION('center_axis',(0.,0.,-1.));
#112241=DIRECTION('ref_axis',(-1.,0.,0.));
#112242=DIRECTION('center_axis',(0.,0.,1.));
#112243=DIRECTION('ref_axis',(1.,0.,0.));
#112244=DIRECTION('',(0.,0.,1.));
#112245=DIRECTION('center_axis',(0.,0.,1.));
#112246=DIRECTION('ref_axis',(1.,0.,0.));
#112247=DIRECTION('center_axis',(0.,0.,1.));
#112248=DIRECTION('ref_axis',(1.,0.,0.));
#112249=DIRECTION('center_axis',(0.,0.,1.));
#112250=DIRECTION('ref_axis',(1.,0.,0.));
#112251=DIRECTION('center_axis',(0.,0.,-1.));
#112252=DIRECTION('ref_axis',(-1.,0.,0.));
#112253=DIRECTION('center_axis',(0.,0.,1.));
#112254=DIRECTION('ref_axis',(1.,0.,0.));
#112255=DIRECTION('',(0.,0.,-1.));
#112256=DIRECTION('center_axis',(0.,0.,1.));
#112257=DIRECTION('ref_axis',(1.,0.,0.));
#112258=DIRECTION('center_axis',(0.,0.,-1.));
#112259=DIRECTION('ref_axis',(-1.,0.,0.));
#112260=DIRECTION('center_axis',(0.,0.,1.));
#112261=DIRECTION('ref_axis',(1.,0.,0.));
#112262=DIRECTION('',(0.,0.,1.));
#112263=DIRECTION('center_axis',(0.,0.,1.));
#112264=DIRECTION('ref_axis',(1.,0.,0.));
#112265=DIRECTION('center_axis',(0.,0.,1.));
#112266=DIRECTION('ref_axis',(1.,0.,0.));
#112267=DIRECTION('center_axis',(0.,0.,1.));
#112268=DIRECTION('ref_axis',(1.,0.,0.));
#112269=DIRECTION('center_axis',(0.,0.,-1.));
#112270=DIRECTION('ref_axis',(-1.,0.,0.));
#112271=DIRECTION('center_axis',(0.,0.,1.));
#112272=DIRECTION('ref_axis',(1.,0.,0.));
#112273=DIRECTION('',(0.,0.,-1.));
#112274=DIRECTION('center_axis',(0.,0.,1.));
#112275=DIRECTION('ref_axis',(1.,0.,0.));
#112276=DIRECTION('center_axis',(0.,0.,-1.));
#112277=DIRECTION('ref_axis',(-1.,0.,0.));
#112278=DIRECTION('center_axis',(0.,0.,1.));
#112279=DIRECTION('ref_axis',(1.,0.,0.));
#112280=DIRECTION('',(0.,0.,1.));
#112281=DIRECTION('center_axis',(0.,0.,1.));
#112282=DIRECTION('ref_axis',(1.,0.,0.));
#112283=DIRECTION('center_axis',(0.,0.,1.));
#112284=DIRECTION('ref_axis',(1.,0.,0.));
#112285=DIRECTION('center_axis',(0.,0.,1.));
#112286=DIRECTION('ref_axis',(1.,0.,0.));
#112287=DIRECTION('center_axis',(0.,0.,-1.));
#112288=DIRECTION('ref_axis',(-1.,0.,0.));
#112289=DIRECTION('center_axis',(0.,0.,-1.));
#112290=DIRECTION('ref_axis',(-1.,0.,0.));
#112291=DIRECTION('center_axis',(0.,0.,-1.));
#112292=DIRECTION('ref_axis',(-1.,0.,0.));
#112293=DIRECTION('center_axis',(-1.22464679914735E-16,-1.,0.));
#112294=DIRECTION('ref_axis',(1.,-1.22464679914735E-16,0.));
#112295=DIRECTION('center_axis',(0.,0.,1.));
#112296=DIRECTION('ref_axis',(-1.,0.,0.));
#112297=DIRECTION('center_axis',(0.,0.,-1.));
#112298=DIRECTION('ref_axis',(-1.,0.,0.));
#112299=DIRECTION('center_axis',(0.,0.,-1.));
#112300=DIRECTION('ref_axis',(-1.,0.,0.));
#112301=DIRECTION('center_axis',(-1.22464679914735E-16,-1.,0.));
#112302=DIRECTION('ref_axis',(1.,-1.22464679914735E-16,0.));
#112303=DIRECTION('center_axis',(0.,0.,1.));
#112304=DIRECTION('ref_axis',(-1.,0.,0.));
#112305=DIRECTION('center_axis',(0.,0.,1.));
#112306=DIRECTION('ref_axis',(-1.,0.,0.));
#112307=DIRECTION('center_axis',(0.,0.,1.));
#112308=DIRECTION('ref_axis',(1.,0.,0.));
#112309=DIRECTION('center_axis',(0.,0.,-1.));
#112310=DIRECTION('ref_axis',(-1.,0.,0.));
#112311=DIRECTION('',(0.,0.,-1.));
#112312=DIRECTION('center_axis',(0.,0.,1.));
#112313=DIRECTION('ref_axis',(1.,0.,0.));
#112314=DIRECTION('',(0.,0.,1.));
#112315=DIRECTION('center_axis',(0.,0.,1.));
#112316=DIRECTION('ref_axis',(-1.,0.,0.));
#112317=DIRECTION('center_axis',(0.,0.,-1.));
#112318=DIRECTION('ref_axis',(-1.,0.,0.));
#112319=DIRECTION('center_axis',(0.,0.,-1.));
#112320=DIRECTION('ref_axis',(-1.,0.,0.));
#112321=DIRECTION('center_axis',(0.,0.,-1.));
#112322=DIRECTION('ref_axis',(-1.,0.,0.));
#112323=DIRECTION('center_axis',(0.,0.,-1.));
#112324=DIRECTION('ref_axis',(-1.,0.,0.));
#112325=DIRECTION('center_axis',(-1.22464679914735E-16,-1.,0.));
#112326=DIRECTION('ref_axis',(1.,-1.22464679914735E-16,0.));
#112327=DIRECTION('center_axis',(0.,0.,1.));
#112328=DIRECTION('ref_axis',(-1.,0.,0.));
#112329=DIRECTION('center_axis',(0.,0.,1.));
#112330=DIRECTION('ref_axis',(-1.,0.,0.));
#112331=DIRECTION('center_axis',(0.,0.,-1.));
#112332=DIRECTION('ref_axis',(-1.,0.,0.));
#112333=DIRECTION('center_axis',(0.,0.,-1.));
#112334=DIRECTION('ref_axis',(-1.,0.,0.));
#112335=DIRECTION('center_axis',(0.,0.,-1.));
#112336=DIRECTION('ref_axis',(-1.,0.,0.));
#112337=DIRECTION('center_axis',(-1.22464679914735E-16,-1.,0.));
#112338=DIRECTION('ref_axis',(1.,-1.22464679914735E-16,0.));
#112339=DIRECTION('center_axis',(0.,0.,1.));
#112340=DIRECTION('ref_axis',(-1.,0.,0.));
#112341=DIRECTION('center_axis',(0.,0.,1.));
#112342=DIRECTION('ref_axis',(1.,0.,0.));
#112343=DIRECTION('center_axis',(0.,0.,-1.));
#112344=DIRECTION('ref_axis',(-1.,0.,0.));
#112345=DIRECTION('',(0.,0.,-1.));
#112346=DIRECTION('center_axis',(0.,0.,1.));
#112347=DIRECTION('ref_axis',(1.,0.,0.));
#112348=DIRECTION('',(0.,0.,1.));
#112349=DIRECTION('center_axis',(0.,0.,-1.));
#112350=DIRECTION('ref_axis',(-1.,0.,0.));
#112351=DIRECTION('center_axis',(0.,0.,-1.));
#112352=DIRECTION('ref_axis',(-1.,0.,0.));
#112353=DIRECTION('center_axis',(0.,0.,-1.));
#112354=DIRECTION('ref_axis',(-1.,0.,0.));
#112355=DIRECTION('center_axis',(0.,0.,1.));
#112356=DIRECTION('ref_axis',(1.,0.,0.));
#112357=DIRECTION('center_axis',(0.,0.,-1.));
#112358=DIRECTION('ref_axis',(-1.,0.,0.));
#112359=DIRECTION('',(0.,0.,1.));
#112360=DIRECTION('center_axis',(0.,0.,-1.));
#112361=DIRECTION('ref_axis',(-1.,0.,0.));
#112362=DIRECTION('center_axis',(0.,0.,1.));
#112363=DIRECTION('ref_axis',(1.,0.,0.));
#112364=DIRECTION('center_axis',(0.,0.,-1.));
#112365=DIRECTION('ref_axis',(-1.,0.,0.));
#112366=DIRECTION('',(0.,0.,-1.));
#112367=DIRECTION('center_axis',(0.,0.,-1.));
#112368=DIRECTION('ref_axis',(-1.,0.,0.));
#112369=DIRECTION('center_axis',(0.,0.,-1.));
#112370=DIRECTION('ref_axis',(-1.,0.,0.));
#112371=DIRECTION('center_axis',(0.,0.,-1.));
#112372=DIRECTION('ref_axis',(-1.,0.,0.));
#112373=DIRECTION('center_axis',(-1.40816906889909E-16,1.4081690688991E-16,
-1.));
#112374=DIRECTION('ref_axis',(0.,1.,1.20114286872534E-16));
#112375=DIRECTION('center_axis',(-1.40816906889909E-16,1.4081690688991E-16,
-1.));
#112376=DIRECTION('ref_axis',(3.27616581394039E-33,1.,1.4081690688991E-16));
#112377=DIRECTION('center_axis',(0.99999996667151,0.00025818012795372,-1.60069213043897E-16));
#112378=DIRECTION('ref_axis',(-0.00025818012795372,0.99999996667151,1.41824142545828E-33));
#112379=DIRECTION('center_axis',(1.4081690688991E-16,0.,1.));
#112380=DIRECTION('ref_axis',(-1.,-4.05186995067197E-12,1.4081690688991E-16));
#112381=DIRECTION('center_axis',(0.99999996667151,-0.000258180127974661,
-1.33391010869915E-16));
#112382=DIRECTION('ref_axis',(0.000258180127974661,0.99999996667151,-9.76420164963656E-34));
#112383=DIRECTION('center_axis',(-1.40816906889909E-16,1.4081690688991E-16,
-1.));
#112384=DIRECTION('ref_axis',(0.,1.,1.12832121675104E-16));
#112385=DIRECTION('center_axis',(-1.4081690688991E-16,0.,-1.));
#112386=DIRECTION('ref_axis',(1.,4.31477076290321E-12,-1.4081690688991E-16));
#112387=DIRECTION('center_axis',(0.999999970597889,0.000242495818320685,
-1.46730112533024E-16));
#112388=DIRECTION('ref_axis',(-0.000242495818320685,0.999999970597889,8.35021668118118E-34));
#112389=DIRECTION('center_axis',(1.40816906889909E-16,-1.4081690688991E-16,
1.));
#112390=DIRECTION('ref_axis',(9.00257646208047E-12,1.,1.40816906888643E-16));
#112391=DIRECTION('center_axis',(0.999999970597889,-0.000242495818341616,
-1.73408314811756E-16));
#112392=DIRECTION('ref_axis',(0.000242495818341616,0.999999970597889,9.96645830604188E-34));
#112393=DIRECTION('center_axis',(-2.81633813779821E-16,0.,-1.));
#112394=DIRECTION('ref_axis',(-1.,0.,2.40228573745067E-16));
#112395=DIRECTION('center_axis',(-2.81633813779821E-16,0.,-1.));
#112396=DIRECTION('ref_axis',(-1.,0.,2.81633813779821E-16));
#112397=DIRECTION('center_axis',(-0.00025818012796419,0.99999996667151,
7.670762046674E-19));
#112398=DIRECTION('ref_axis',(-0.99999996667151,-0.00025818012796419,4.77318454276342E-36));
#112399=DIRECTION('center_axis',(1.4081690688991E-16,0.,1.));
#112400=DIRECTION('ref_axis',(-1.,-2.90079071874061E-12,1.4081690688991E-16));
#112401=DIRECTION('center_axis',(0.00025818012796419,0.99999996667151,-7.670762046674E-19));
#112402=DIRECTION('ref_axis',(-0.99999996667151,0.00025818012796419,4.77318454276342E-36));
#112403=DIRECTION('center_axis',(-2.81633813779821E-16,0.,-1.));
#112404=DIRECTION('ref_axis',(-1.,0.,2.25664243350207E-16));
#112405=DIRECTION('center_axis',(-1.4081690688991E-16,0.,-1.));
#112406=DIRECTION('ref_axis',(1.,0.,-1.4081690688991E-16));
#112407=DIRECTION('center_axis',(-0.000242495818331158,0.999999970597889,
0.));
#112408=DIRECTION('ref_axis',(-0.999999970597889,-0.000242495818331158,
0.));
#112409=DIRECTION('center_axis',(2.81633813779821E-16,0.,1.));
#112410=DIRECTION('ref_axis',(-1.,-9.2414964569798E-12,2.81633813779821E-16));
#112411=DIRECTION('center_axis',(0.00024249581833115,0.999999970597889,
-1.33391011393658E-17));
#112412=DIRECTION('ref_axis',(-0.999999970597889,0.00024249581833115,2.11314776580936E-36));
#112413=DIRECTION('center_axis',(-1.4081690688991E-16,0.,-1.));
#112414=DIRECTION('ref_axis',(1.,0.,-1.4081690688991E-16));
#112415=DIRECTION('center_axis',(-1.4081690688991E-16,0.,-1.));
#112416=DIRECTION('ref_axis',(-1.,0.,1.20729796120972E-16));
#112417=DIRECTION('center_axis',(-1.4081690688991E-16,0.,-1.));
#112418=DIRECTION('ref_axis',(-1.,0.,1.4081690688991E-16));
#112419=DIRECTION('center_axis',(-1.22464679914735E-16,-1.,1.7245097428856E-32));
#112420=DIRECTION('ref_axis',(1.,-1.22464679914735E-16,-1.50912245151216E-16));
#112421=DIRECTION('center_axis',(1.4081690688991E-16,0.,1.));
#112422=DIRECTION('ref_axis',(-1.,0.,1.4081690688991E-16));
#112423=DIRECTION('center_axis',(1.4081690688991E-16,0.,1.));
#112424=DIRECTION('ref_axis',(-1.,0.,1.4081690688991E-16));
#112425=DIRECTION('center_axis',(-1.4081690688991E-16,0.,-1.));
#112426=DIRECTION('ref_axis',(-1.,0.,1.20546251308204E-16));
#112427=DIRECTION('center_axis',(-1.4081690688991E-16,0.,-1.));
#112428=DIRECTION('ref_axis',(1.,0.,-1.4081690688991E-16));
#112429=DIRECTION('center_axis',(-1.22464679914735E-16,-1.,1.7245097428856E-32));
#112430=DIRECTION('ref_axis',(1.,-1.22464679914735E-16,-1.50682814135255E-16));
#112431=DIRECTION('center_axis',(1.4081690688991E-16,0.,1.));
#112432=DIRECTION('ref_axis',(-1.,0.,1.40816906889911E-16));
#112433=DIRECTION('center_axis',(-1.4081690688991E-16,0.,-1.));
#112434=DIRECTION('ref_axis',(-1.,0.,1.10673987086231E-16));
#112435=DIRECTION('center_axis',(-1.4081690688991E-16,0.,-1.));
#112436=DIRECTION('ref_axis',(-1.,0.,1.4081690688991E-16));
#112437=DIRECTION('center_axis',(-1.22464679914735E-16,-1.,1.7245097428856E-32));
#112438=DIRECTION('ref_axis',(1.,-1.22464679914735E-16,-1.38342483857788E-16));
#112439=DIRECTION('center_axis',(1.4081690688991E-16,0.,1.));
#112440=DIRECTION('ref_axis',(-1.,0.,1.40816906889911E-16));
#112441=DIRECTION('center_axis',(1.4081690688991E-16,0.,1.));
#112442=DIRECTION('ref_axis',(-1.,0.,1.40816906889911E-16));
#112443=DIRECTION('center_axis',(-1.4081690688991E-16,0.,-1.));
#112444=DIRECTION('ref_axis',(-1.,0.,1.10519724968194E-16));
#112445=DIRECTION('center_axis',(-1.4081690688991E-16,0.,-1.));
#112446=DIRECTION('ref_axis',(1.,0.,-1.4081690688991E-16));
#112447=DIRECTION('center_axis',(-1.22464679914735E-16,-1.,1.7245097428856E-32));
#112448=DIRECTION('ref_axis',(1.,-1.22464679914735E-16,-1.38149656210243E-16));
#112449=DIRECTION('center_axis',(1.4081690688991E-16,0.,1.));
#112450=DIRECTION('ref_axis',(-1.,0.,1.40816906889911E-16));
#112451=DIRECTION('center_axis',(-1.4081690688991E-16,0.,-1.));
#112452=DIRECTION('ref_axis',(-1.,0.,1.4081690688991E-16));
#112453=DIRECTION('center_axis',(-1.4081690688991E-16,0.,-1.));
#112454=DIRECTION('ref_axis',(-1.,0.,1.4081690688991E-16));
#112455=DIRECTION('',(1.4081690688991E-16,0.,1.));
#112456=DIRECTION('center_axis',(-1.4081690688991E-16,0.,-1.));
#112457=DIRECTION('ref_axis',(-1.,0.,1.4081690688991E-16));
#112458=DIRECTION('center_axis',(-1.4081690688991E-16,0.,-1.));
#112459=DIRECTION('ref_axis',(-1.,0.,1.4081690688991E-16));
#112460=DIRECTION('',(-0.529919264233199,6.48963930749707E-17,0.84804809615643));
#112461=DIRECTION('center_axis',(1.4081690688991E-16,0.,1.));
#112462=DIRECTION('ref_axis',(1.,0.,-1.4081690688991E-16));
#112463=DIRECTION('center_axis',(-1.4081690688991E-16,0.,-1.));
#112464=DIRECTION('ref_axis',(1.,0.,-1.4081690688991E-16));
#112465=DIRECTION('',(-0.529924202082878,-4.6420044039426E-6,-0.848045010612808));
#112466=DIRECTION('center_axis',(-1.4081690688991E-16,0.,-1.));
#112467=DIRECTION('ref_axis',(1.,0.,-1.4081690688991E-16));
#112468=DIRECTION('',(0.527020736635428,-0.0553967790670814,0.848045010612788));
#112469=DIRECTION('center_axis',(-1.4081690688991E-16,0.,-1.));
#112470=DIRECTION('ref_axis',(1.,6.21724893790088E-15,-1.4081690688991E-16));
#112471=DIRECTION('',(-0.527021707078575,0.0553875459170483,-0.848045010612805));
#112472=DIRECTION('center_axis',(-1.4081690688991E-16,0.,-1.));
#112473=DIRECTION('ref_axis',(1.,0.,-1.4081690688991E-16));
#112474=DIRECTION('',(0.518343121711168,-0.11018197742578,0.848045010612801));
#112475=DIRECTION('center_axis',(-1.4081690688991E-16,0.,-1.));
#112476=DIRECTION('ref_axis',(1.,1.24344978758018E-14,-1.4081690688991E-16));
#112477=DIRECTION('',(-0.51834505196515,0.110172896294841,-0.848045010612793));
#112478=DIRECTION('center_axis',(-1.4081690688991E-16,0.,-1.));
#112479=DIRECTION('ref_axis',(1.,0.,-1.4081690688991E-16));
#112480=DIRECTION('',(0.50398643107519,-0.163759998982733,0.848045010612802));
#112481=DIRECTION('center_axis',(-1.4081690688991E-16,0.,-1.));
#112482=DIRECTION('ref_axis',(1.,0.,-1.4081690688991E-16));
#112483=DIRECTION('',(-0.503989299991689,0.163751169365661,-0.848045010612801));
#112484=DIRECTION('center_axis',(-1.4081690688991E-16,0.,-1.));
#112485=DIRECTION('ref_axis',(1.,0.,-1.4081690688991E-16));
#112486=DIRECTION('',(0.484107959634419,-0.215543831721857,0.848045010612797));
#112487=DIRECTION('center_axis',(-1.4081690688991E-16,0.,-1.));
#112488=DIRECTION('ref_axis',(1.,4.79616346638068E-14,-1.4081690688991E-16));
#112489=DIRECTION('',(-0.484111735780994,0.215535350357782,-0.848045010612798));
#112490=DIRECTION('center_axis',(-1.4081690688991E-16,0.,-1.));
#112491=DIRECTION('ref_axis',(1.,8.88178419700125E-16,-1.4081690688991E-16));
#112492=DIRECTION('',(0.458925500081788,-0.26496612113519,0.848045010612793));
#112493=DIRECTION('center_axis',(-1.4081690688991E-16,0.,-1.));
#112494=DIRECTION('ref_axis',(1.,0.,-1.4081690688991E-16));
#112495=DIRECTION('',(-0.458930142086183,0.264958080947708,-0.8480450106128));
#112496=DIRECTION('center_axis',(-1.4081690688991E-16,0.,-1.));
#112497=DIRECTION('ref_axis',(1.,8.88178419700125E-16,-1.4081690688991E-16));
#112498=DIRECTION('',(0.428714956713914,-0.311485386277621,0.848045010612803));
#112499=DIRECTION('center_axis',(-1.4081690688991E-16,0.,-1.));
#112500=DIRECTION('ref_axis',(1.,0.,-1.4081690688991E-16));
#112501=DIRECTION('',(-0.428720413717376,0.311477875356734,-0.848045010612796));
#112502=DIRECTION('center_axis',(-1.4081690688991E-16,0.,-1.));
#112503=DIRECTION('ref_axis',(1.,8.88178419700125E-16,-1.4081690688991E-16));
#112504=DIRECTION('',(0.393807322565914,-0.354591952345506,0.848045010612802));
#112505=DIRECTION('center_axis',(-1.4081690688991E-16,0.,-1.));
#112506=DIRECTION('ref_axis',(1.,0.,-1.4081690688991E-16));
#112507=DIRECTION('',(-0.393813534780369,0.354585052982416,-0.848045010612791));
#112508=DIRECTION('center_axis',(-1.4081690688991E-16,0.,-1.));
#112509=DIRECTION('ref_axis',(1.,8.88178419700125E-16,-1.4081690688991E-16));
#112510=DIRECTION('',(0.354585052982406,-0.39381353478036,0.848045010612799));
#112511=DIRECTION('center_axis',(-1.4081690688991E-16,0.,-1.));
#112512=DIRECTION('ref_axis',(1.,0.,-1.4081690688991E-16));
#112513=DIRECTION('',(-0.354591952345518,0.393807322565912,-0.848045010612799));
#112514=DIRECTION('center_axis',(-1.4081690688991E-16,0.,-1.));
#112515=DIRECTION('ref_axis',(1.,8.88178419700125E-16,-1.4081690688991E-16));
#112516=DIRECTION('',(0.311477875356732,-0.428720413717355,0.848045010612807));
#112517=DIRECTION('center_axis',(-1.4081690688991E-16,0.,-1.));
#112518=DIRECTION('ref_axis',(1.,0.,-1.4081690688991E-16));
#112519=DIRECTION('',(-0.311485386277638,0.428714956713914,-0.848045010612796));
#112520=DIRECTION('center_axis',(-1.4081690688991E-16,0.,-1.));
#112521=DIRECTION('ref_axis',(1.,0.,-1.4081690688991E-16));
#112522=DIRECTION('',(0.264958080947704,-0.458930142086175,0.848045010612805));
#112523=DIRECTION('center_axis',(-1.4081690688991E-16,0.,-1.));
#112524=DIRECTION('ref_axis',(1.,0.,-1.4081690688991E-16));
#112525=DIRECTION('',(-0.264966121135182,0.45892550008177,-0.848045010612805));
#112526=DIRECTION('center_axis',(-1.4081690688991E-16,0.,-1.));
#112527=DIRECTION('ref_axis',(1.,0.,-1.4081690688991E-16));
#112528=DIRECTION('',(0.215535350357774,-0.484111735780989,0.848045010612803));
#112529=DIRECTION('center_axis',(-1.4081690688991E-16,0.,-1.));
#112530=DIRECTION('ref_axis',(1.,0.,-1.4081690688991E-16));
#112531=DIRECTION('',(-0.215543831721856,0.484107959634404,-0.848045010612807));
#112532=DIRECTION('center_axis',(-1.4081690688991E-16,0.,-1.));
#112533=DIRECTION('ref_axis',(1.,0.,-1.4081690688991E-16));
#112534=DIRECTION('',(0.163751169365657,-0.503989299991686,0.848045010612804));
#112535=DIRECTION('center_axis',(-1.4081690688991E-16,0.,-1.));
#112536=DIRECTION('ref_axis',(1.,0.,-1.4081690688991E-16));
#112537=DIRECTION('',(-0.163759998982741,0.503986431075192,-0.8480450106128));
#112538=DIRECTION('center_axis',(-1.4081690688991E-16,0.,-1.));
#112539=DIRECTION('ref_axis',(1.,0.,-1.4081690688991E-16));
#112540=DIRECTION('',(0.110172896294838,-0.518345051965138,0.848045010612801));
#112541=DIRECTION('center_axis',(-1.4081690688991E-16,0.,-1.));
#112542=DIRECTION('ref_axis',(1.,0.,-1.4081690688991E-16));
#112543=DIRECTION('',(-0.110181977425777,0.518343121711181,-0.848045010612794));
#112544=DIRECTION('center_axis',(-1.4081690688991E-16,0.,-1.));
#112545=DIRECTION('ref_axis',(1.,0.,-1.4081690688991E-16));
#112546=DIRECTION('',(0.055387545917043,-0.527021707078587,0.848045010612797));
#112547=DIRECTION('center_axis',(-1.4081690688991E-16,0.,-1.));
#112548=DIRECTION('ref_axis',(1.,0.,-1.4081690688991E-16));
#112549=DIRECTION('',(-0.0553967790670791,0.527020736635425,-0.84804501061279));
#112550=DIRECTION('center_axis',(-1.4081690688991E-16,0.,-1.));
#112551=DIRECTION('ref_axis',(1.,0.,-1.4081690688991E-16));
#112552=DIRECTION('',(-4.64200440569703E-6,-0.529924202082903,0.848045010612792));
#112553=DIRECTION('center_axis',(-1.4081690688991E-16,0.,-1.));
#112554=DIRECTION('ref_axis',(1.,0.,-1.4081690688991E-16));
#112555=DIRECTION('',(-4.6420044022913E-6,0.529924202082884,-0.848045010612804));
#112556=DIRECTION('center_axis',(-1.4081690688991E-16,0.,-1.));
#112557=DIRECTION('ref_axis',(1.,0.,-1.4081690688991E-16));
#112558=DIRECTION('',(-0.0553967790670824,-0.527020736635424,0.84804501061279));
#112559=DIRECTION('center_axis',(-1.4081690688991E-16,0.,-1.));
#112560=DIRECTION('ref_axis',(1.,0.,-1.4081690688991E-16));
#112561=DIRECTION('',(0.0553875459170473,0.527021707078581,-0.848045010612801));
#112562=DIRECTION('center_axis',(-1.4081690688991E-16,0.,-1.));
#112563=DIRECTION('ref_axis',(1.,0.,-1.4081690688991E-16));
#112564=DIRECTION('',(-0.110181977425775,-0.518343121711175,0.848045010612798));
#112565=DIRECTION('center_axis',(-1.4081690688991E-16,0.,-1.));
#112566=DIRECTION('ref_axis',(1.,0.,-1.4081690688991E-16));
#112567=DIRECTION('',(0.110172896294838,0.518345051965151,-0.848045010612793));
#112568=DIRECTION('center_axis',(-1.4081690688991E-16,0.,-1.));
#112569=DIRECTION('ref_axis',(1.,0.,-1.4081690688991E-16));
#112570=DIRECTION('',(-0.163759998982731,-0.503986431075193,0.848045010612801));
#112571=DIRECTION('center_axis',(-1.4081690688991E-16,0.,-1.));
#112572=DIRECTION('ref_axis',(1.,0.,-1.4081690688991E-16));
#112573=DIRECTION('',(0.163751169365665,0.503989299991695,-0.848045010612797));
#112574=DIRECTION('center_axis',(-1.4081690688991E-16,0.,-1.));
#112575=DIRECTION('ref_axis',(1.,0.,-1.4081690688991E-16));
#112576=DIRECTION('',(-0.215543831721855,-0.484107959634416,0.848045010612799));
#112577=DIRECTION('center_axis',(-1.4081690688991E-16,0.,-1.));
#112578=DIRECTION('ref_axis',(1.,0.,-1.4081690688991E-16));
#112579=DIRECTION('',(0.215535350357775,0.484111735780992,-0.848045010612802));
#112580=DIRECTION('center_axis',(-1.4081690688991E-16,0.,-1.));
#112581=DIRECTION('ref_axis',(1.,-4.44089209850063E-15,-1.4081690688991E-16));
#112582=DIRECTION('',(-0.264966121135187,-0.458925500081781,0.848045010612798));
#112583=DIRECTION('center_axis',(-1.4081690688991E-16,0.,-1.));
#112584=DIRECTION('ref_axis',(1.,0.,-1.4081690688991E-16));
#112585=DIRECTION('',(0.264958080947722,0.458930142086184,-0.848045010612795));
#112586=DIRECTION('center_axis',(-1.4081690688991E-16,0.,-1.));
#112587=DIRECTION('ref_axis',(1.,0.,-1.4081690688991E-16));
#112588=DIRECTION('',(-0.31148538627764,-0.428714956713913,0.848045010612796));
#112589=DIRECTION('center_axis',(-1.4081690688991E-16,0.,-1.));
#112590=DIRECTION('ref_axis',(1.,2.01438865587988E-12,-1.4081690688991E-16));
#112591=DIRECTION('',(0.311477875356739,0.428720413717396,-0.848045010612783));
#112592=DIRECTION('center_axis',(-1.4081690688991E-16,0.,-1.));
#112593=DIRECTION('ref_axis',(1.,0.,-1.4081690688991E-16));
#112594=DIRECTION('',(-0.354591952345506,-0.393807322565927,0.848045010612796));
#112595=DIRECTION('center_axis',(-1.4081690688991E-16,0.,-1.));
#112596=DIRECTION('ref_axis',(1.,0.,-1.4081690688991E-16));
#112597=DIRECTION('',(0.354585052982408,0.393813534780362,-0.848045010612797));
#112598=DIRECTION('center_axis',(-1.4081690688991E-16,0.,-1.));
#112599=DIRECTION('ref_axis',(1.,0.,-1.4081690688991E-16));
#112600=DIRECTION('',(-0.393813534780346,-0.354585052982406,0.848045010612805));
#112601=DIRECTION('center_axis',(-1.4081690688991E-16,0.,-1.));
#112602=DIRECTION('ref_axis',(1.,-2.20534701611541E-12,-1.4081690688991E-16));
#112603=DIRECTION('',(0.393807322565923,0.354591952345502,-0.8480450106128));
#112604=DIRECTION('center_axis',(-1.4081690688991E-16,0.,-1.));
#112605=DIRECTION('ref_axis',(1.,1.15463194561016E-14,-1.4081690688991E-16));
#112606=DIRECTION('',(-0.428720413717367,-0.311477875356727,0.848045010612803));
#112607=DIRECTION('center_axis',(-1.4081690688991E-16,0.,-1.));
#112608=DIRECTION('ref_axis',(1.,0.,-1.4081690688991E-16));
#112609=DIRECTION('',(0.428714956713905,0.311485386277624,-0.848045010612805));
#112610=DIRECTION('center_axis',(-1.4081690688991E-16,0.,-1.));
#112611=DIRECTION('ref_axis',(1.,0.,-1.4081690688991E-16));
#112612=DIRECTION('',(-0.458930142086187,-0.264958080947698,0.848045010612801));
#112613=DIRECTION('center_axis',(-1.4081690688991E-16,0.,-1.));
#112614=DIRECTION('ref_axis',(1.,0.,-1.4081690688991E-16));
#112615=DIRECTION('',(0.458925500081769,0.264966121135188,-0.848045010612804));
#112616=DIRECTION('center_axis',(-1.4081690688991E-16,0.,-1.));
#112617=DIRECTION('ref_axis',(1.,0.,-1.4081690688991E-16));
#112618=DIRECTION('',(-0.484111735781008,-0.21553535035777,0.848045010612794));
#112619=DIRECTION('center_axis',(-1.4081690688991E-16,0.,-1.));
#112620=DIRECTION('ref_axis',(1.,0.,-1.4081690688991E-16));
#112621=DIRECTION('',(0.484107959634402,0.215543831721842,-0.848045010612811));
#112622=DIRECTION('center_axis',(-1.4081690688991E-16,0.,-1.));
#112623=DIRECTION('ref_axis',(1.,0.,-1.4081690688991E-16));
#112624=DIRECTION('',(-0.503989299991702,-0.163751169365651,0.848045010612795));
#112625=DIRECTION('center_axis',(-1.4081690688991E-16,0.,-1.));
#112626=DIRECTION('ref_axis',(1.,0.,-1.4081690688991E-16));
#112627=DIRECTION('',(0.503986431075198,0.163759998982739,-0.848045010612796));
#112628=DIRECTION('center_axis',(-1.4081690688991E-16,0.,-1.));
#112629=DIRECTION('ref_axis',(1.,0.,-1.4081690688991E-16));
#112630=DIRECTION('',(-0.518345051965132,-0.110172896294837,0.848045010612804));
#112631=DIRECTION('center_axis',(-1.4081690688991E-16,0.,-1.));
#112632=DIRECTION('ref_axis',(1.,0.,-1.4081690688991E-16));
#112633=DIRECTION('',(0.518343121711172,0.110181977425774,-0.8480450106128));
#112634=DIRECTION('center_axis',(-1.4081690688991E-16,0.,-1.));
#112635=DIRECTION('ref_axis',(1.,0.,-1.4081690688991E-16));
#112636=DIRECTION('',(-0.527021707078582,-0.0553875459170411,0.848045010612801));
#112637=DIRECTION('center_axis',(-1.4081690688991E-16,0.,-1.));
#112638=DIRECTION('ref_axis',(1.,0.,-1.4081690688991E-16));
#112639=DIRECTION('',(0.527020736635406,0.0553967790670803,-0.848045010612802));
#112640=DIRECTION('center_axis',(-1.4081690688991E-16,0.,-1.));
#112641=DIRECTION('ref_axis',(1.,0.,-1.4081690688991E-16));
#112642=DIRECTION('',(-0.529924202082894,4.64200440404571E-6,0.848045010612798));
#112643=DIRECTION('',(-0.529919264233196,-6.48963930749704E-17,0.848048096156432));
#112644=DIRECTION('',(0.529924202082894,4.64200440394251E-6,-0.848045010612798));
#112645=DIRECTION('center_axis',(-1.4081690688991E-16,0.,-1.));
#112646=DIRECTION('ref_axis',(1.,0.,-1.4081690688991E-16));
#112647=DIRECTION('',(-0.527020736635415,0.0553967790670848,0.848045010612796));
#112648=DIRECTION('center_axis',(-1.4081690688991E-16,0.,-1.));
#112649=DIRECTION('ref_axis',(1.,0.,-1.4081690688991E-16));
#112650=DIRECTION('',(0.527021707078572,-0.055387545917048,-0.848045010612806));
#112651=DIRECTION('center_axis',(-1.4081690688991E-16,0.,-1.));
#112652=DIRECTION('ref_axis',(1.,0.,-1.4081690688991E-16));
#112653=DIRECTION('',(-0.518343121711156,0.110181977425777,0.848045010612809));
#112654=DIRECTION('center_axis',(-1.4081690688991E-16,0.,-1.));
#112655=DIRECTION('ref_axis',(1.,0.,-1.4081690688991E-16));
#112656=DIRECTION('',(0.518345051965142,-0.110172896294836,-0.848045010612799));
#112657=DIRECTION('center_axis',(-1.4081690688991E-16,0.,-1.));
#112658=DIRECTION('ref_axis',(1.,0.,-1.4081690688991E-16));
#112659=DIRECTION('',(-0.503986431075197,0.163759998982742,0.848045010612796));
#112660=DIRECTION('center_axis',(-1.4081690688991E-16,0.,-1.));
#112661=DIRECTION('ref_axis',(1.,0.,-1.4081690688991E-16));
#112662=DIRECTION('',(0.503989299991692,-0.163751169365662,-0.848045010612799));
#112663=DIRECTION('center_axis',(-1.4081690688991E-16,0.,-1.));
#112664=DIRECTION('ref_axis',(1.,0.,-1.4081690688991E-16));
#112665=DIRECTION('',(-0.484107959634421,0.215543831721864,0.848045010612794));
#112666=DIRECTION('center_axis',(-1.4081690688991E-16,0.,-1.));
#112667=DIRECTION('ref_axis',(1.,0.,-1.4081690688991E-16));
#112668=DIRECTION('',(0.484111735780995,-0.215535350357796,-0.848045010612794));
#112669=DIRECTION('center_axis',(-1.4081690688991E-16,0.,-1.));
#112670=DIRECTION('ref_axis',(1.,0.,-1.4081690688991E-16));
#112671=DIRECTION('',(-0.45892550008179,0.264966121135192,0.848045010612791));
#112672=DIRECTION('center_axis',(-1.4081690688991E-16,0.,-1.));
#112673=DIRECTION('ref_axis',(1.,0.,-1.4081690688991E-16));
#112674=DIRECTION('',(0.458930142086184,-0.264958080947722,-0.848045010612795));
#112675=DIRECTION('center_axis',(-1.4081690688991E-16,0.,-1.));
#112676=DIRECTION('ref_axis',(1.,0.,-1.4081690688991E-16));
#112677=DIRECTION('',(-0.428714956713903,0.311485386277636,0.848045010612802));
#112678=DIRECTION('center_axis',(-1.4081690688991E-16,0.,-1.));
#112679=DIRECTION('ref_axis',(1.,0.,-1.4081690688991E-16));
#112680=DIRECTION('',(0.428720413717366,-0.311477875356733,-0.848045010612801));
#112681=DIRECTION('center_axis',(-1.4081690688991E-16,0.,-1.));
#112682=DIRECTION('ref_axis',(1.,0.,-1.4081690688991E-16));
#112683=DIRECTION('',(-0.393807322565926,0.354591952345518,0.848045010612792));
#112684=DIRECTION('center_axis',(-1.4081690688991E-16,0.,-1.));
#112685=DIRECTION('ref_axis',(1.,0.,-1.4081690688991E-16));
#112686=DIRECTION('',(0.393813534780356,-0.354585052982416,-0.848045010612797));
#112687=DIRECTION('center_axis',(-1.4081690688991E-16,0.,-1.));
#112688=DIRECTION('ref_axis',(1.,0.,-1.4081690688991E-16));
#112689=DIRECTION('',(-0.35458505298241,0.393813534780351,0.848045010612802));
#112690=DIRECTION('center_axis',(-1.4081690688991E-16,0.,-1.));
#112691=DIRECTION('ref_axis',(1.,0.,-1.4081690688991E-16));
#112692=DIRECTION('',(0.354591952345508,-0.393807322565916,-0.848045010612801));
#112693=DIRECTION('center_axis',(-1.4081690688991E-16,0.,-1.));
#112694=DIRECTION('ref_axis',(1.,0.,-1.4081690688991E-16));
#112695=DIRECTION('',(-0.311477875356733,0.428720413717371,0.848045010612799));
#112696=DIRECTION('center_axis',(-1.4081690688991E-16,0.,-1.));
#112697=DIRECTION('ref_axis',(1.,7.47846229387506E-12,-1.4081690688991E-16));
#112698=DIRECTION('',(0.311485386277631,-0.428714956713909,-0.848045010612801));
#112699=DIRECTION('center_axis',(-1.4081690688991E-16,0.,-1.));
#112700=DIRECTION('ref_axis',(1.,0.,-1.4081690688991E-16));
#112701=DIRECTION('',(-0.264958080947707,0.458930142086206,0.848045010612788));
#112702=DIRECTION('center_axis',(-1.4081690688991E-16,0.,-1.));
#112703=DIRECTION('ref_axis',(1.,3.83604259468484E-12,-1.4081690688991E-16));
#112704=DIRECTION('',(0.26496612113518,-0.458925500081792,-0.848045010612794));
#112705=DIRECTION('center_axis',(-1.4081690688991E-16,0.,-1.));
#112706=DIRECTION('ref_axis',(1.,-3.01980662698043E-14,-1.4081690688991E-16));
#112707=DIRECTION('',(-0.215535350357775,0.484111735780992,0.848045010612802));
#112708=DIRECTION('center_axis',(-1.4081690688991E-16,0.,-1.));
#112709=DIRECTION('ref_axis',(1.,-5.89750470680883E-12,-1.4081690688991E-16));
#112710=DIRECTION('',(0.21554383172186,-0.484107959634426,-0.848045010612793));
#112711=DIRECTION('center_axis',(-1.4081690688991E-16,0.,-1.));
#112712=DIRECTION('ref_axis',(1.,1.06581410364015E-14,-1.4081690688991E-16));
#112713=DIRECTION('',(-0.163751169365653,0.5039892999917,0.848045010612796));
#112714=DIRECTION('center_axis',(-1.4081690688991E-16,0.,-1.));
#112715=DIRECTION('ref_axis',(1.,-6.04050143238055E-12,-1.4081690688991E-16));
#112716=DIRECTION('',(0.163759998982731,-0.503986431075193,-0.848045010612801));
#112717=DIRECTION('center_axis',(-1.4081690688991E-16,0.,-1.));
#112718=DIRECTION('ref_axis',(1.,1.06581410364015E-14,-1.4081690688991E-16));
#112719=DIRECTION('',(-0.110172896294832,0.518345051965141,0.848045010612799));
#112720=DIRECTION('center_axis',(-1.4081690688991E-16,0.,-1.));
#112721=DIRECTION('ref_axis',(1.,-6.18438633637197E-12,-1.4081690688991E-16));
#112722=DIRECTION('',(0.11018197742577,-0.518343121711171,-0.848045010612801));
#112723=DIRECTION('center_axis',(-1.4081690688991E-16,0.,-1.));
#112724=DIRECTION('ref_axis',(1.,1.06581410364015E-14,-1.4081690688991E-16));
#112725=DIRECTION('',(-0.0553875459170391,0.527021707078581,0.848045010612801));
#112726=DIRECTION('center_axis',(-1.4081690688991E-16,0.,-1.));
#112727=DIRECTION('ref_axis',(1.,2.1094237467878E-12,-1.4081690688991E-16));
#112728=DIRECTION('',(0.0553967790670773,-0.527020736635409,-0.8480450106128));
#112729=DIRECTION('center_axis',(-1.4081690688991E-16,0.,-1.));
#112730=DIRECTION('ref_axis',(1.,-3.37507799486048E-14,-1.4081690688991E-16));
#112731=DIRECTION('',(4.64200440982517E-6,0.529924202082893,0.848045010612798));
#112732=DIRECTION('',(4.64200439836961E-6,-0.529924202082884,-0.848045010612804));
#112733=DIRECTION('center_axis',(-1.4081690688991E-16,0.,-1.));
#112734=DIRECTION('ref_axis',(1.,-3.37507799486048E-14,-1.4081690688991E-16));
#112735=DIRECTION('',(0.0553967790670853,0.527020736635434,0.848045010612784));
#112736=DIRECTION('center_axis',(-1.4081690688991E-16,0.,-1.));
#112737=DIRECTION('ref_axis',(1.,0.,-1.4081690688991E-16));
#112738=DIRECTION('',(-0.0553875459170506,-0.527021707078581,-0.848045010612801));
#112739=DIRECTION('center_axis',(-1.4081690688991E-16,0.,-1.));
#112740=DIRECTION('ref_axis',(1.,1.06581410364015E-14,-1.4081690688991E-16));
#112741=DIRECTION('',(0.110181977425778,0.518343121711174,0.848045010612798));
#112742=DIRECTION('center_axis',(-1.4081690688991E-16,0.,-1.));
#112743=DIRECTION('ref_axis',(1.,0.,-1.4081690688991E-16));
#112744=DIRECTION('',(-0.110172896294837,-0.518345051965147,-0.848045010612795));
#112745=DIRECTION('center_axis',(-1.4081690688991E-16,0.,-1.));
#112746=DIRECTION('ref_axis',(1.,0.,-1.4081690688991E-16));
#112747=DIRECTION('',(0.163759998982748,0.503986431075194,0.848045010612797));
#112748=DIRECTION('center_axis',(-1.4081690688991E-16,0.,-1.));
#112749=DIRECTION('ref_axis',(1.,0.,-1.4081690688991E-16));
#112750=DIRECTION('',(-0.163751169365666,-0.503989299991698,-0.848045010612795));
#112751=DIRECTION('center_axis',(-1.4081690688991E-16,0.,-1.));
#112752=DIRECTION('ref_axis',(1.,-3.5527136788005E-14,-1.4081690688991E-16));
#112753=DIRECTION('',(0.215543831721856,0.484107959634404,0.848045010612807));
#112754=DIRECTION('center_axis',(-1.4081690688991E-16,0.,-1.));
#112755=DIRECTION('ref_axis',(1.,2.34923192010683E-12,-1.4081690688991E-16));
#112756=DIRECTION('',(-0.215535350357785,-0.484111735780998,-0.848045010612796));
#112757=DIRECTION('center_axis',(-1.4081690688991E-16,0.,-1.));
#112758=DIRECTION('ref_axis',(1.,-3.5527136788005E-14,-1.4081690688991E-16));
#112759=DIRECTION('',(0.264966121135194,0.458925500081769,0.848045010612802));
#112760=DIRECTION('center_axis',(-1.4081690688991E-16,0.,-1.));
#112761=DIRECTION('ref_axis',(1.,0.,-1.4081690688991E-16));
#112762=DIRECTION('',(-0.264958080947704,-0.458930142086175,-0.848045010612805));
#112763=DIRECTION('center_axis',(-1.4081690688991E-16,0.,-1.));
#112764=DIRECTION('ref_axis',(1.,-4.2632564145606E-14,-1.4081690688991E-16));
#112765=DIRECTION('',(0.311485386277635,0.428714956713893,0.848045010612808));
#112766=DIRECTION('center_axis',(-1.4081690688991E-16,0.,-1.));
#112767=DIRECTION('ref_axis',(1.,2.44515518943444E-12,-1.4081690688991E-16));
#112768=DIRECTION('',(-0.311477875356743,-0.428720413717361,-0.8480450106128));
#112769=DIRECTION('center_axis',(-1.4081690688991E-16,0.,-1.));
#112770=DIRECTION('ref_axis',(1.,-2.48689957516035E-14,-1.4081690688991E-16));
#112771=DIRECTION('',(0.354591952345522,0.393807322565903,0.848045010612801));
#112772=DIRECTION('center_axis',(-1.4081690688991E-16,0.,-1.));
#112773=DIRECTION('ref_axis',(1.,-4.9862336481965E-12,-1.4081690688991E-16));
#112774=DIRECTION('',(-0.354585052982408,-0.393813534780349,-0.848045010612804));
#112775=DIRECTION('center_axis',(-1.4081690688991E-16,0.,-1.));
#112776=DIRECTION('ref_axis',(1.,0.,-1.4081690688991E-16));
#112777=DIRECTION('',(0.39381353478036,0.354585052982406,0.848045010612799));
#112778=DIRECTION('center_axis',(-1.4081690688991E-16,0.,-1.));
#112779=DIRECTION('ref_axis',(1.,1.27009514017118E-12,-1.4081690688991E-16));
#112780=DIRECTION('',(-0.393807322565912,-0.354591952345518,-0.848045010612799));
#112781=DIRECTION('center_axis',(-1.4081690688991E-16,0.,-1.));
#112782=DIRECTION('ref_axis',(1.,1.33226762955019E-14,-1.4081690688991E-16));
#112783=DIRECTION('',(0.428720413717364,0.311477875356725,0.848045010612805));
#112784=DIRECTION('center_axis',(-1.4081690688991E-16,0.,-1.));
#112785=DIRECTION('ref_axis',(1.,1.29407595750308E-12,-1.4081690688991E-16));
#112786=DIRECTION('',(-0.428714956713912,-0.311485386277633,-0.848045010612799));
#112787=DIRECTION('center_axis',(-1.4081690688991E-16,0.,-1.));
#112788=DIRECTION('ref_axis',(1.,-4.08562073062058E-14,-1.4081690688991E-16));
#112789=DIRECTION('',(0.458930142086183,0.264958080947708,0.8480450106128));
#112790=DIRECTION('center_axis',(-1.4081690688991E-16,0.,-1.));
#112791=DIRECTION('ref_axis',(1.,1.31805677483499E-12,-1.4081690688991E-16));
#112792=DIRECTION('',(-0.458925500081773,-0.264966121135183,-0.848045010612804));
#112793=DIRECTION('center_axis',(-1.4081690688991E-16,0.,-1.));
#112794=DIRECTION('ref_axis',(1.,9.76996261670138E-15,-1.4081690688991E-16));
#112795=DIRECTION('',(0.48411173578099,0.215535350357767,0.848045010612805));
#112796=DIRECTION('center_axis',(-1.4081690688991E-16,0.,-1.));
#112797=DIRECTION('ref_axis',(1.,2.01350047746018E-12,-1.4081690688991E-16));
#112798=DIRECTION('',(-0.484107959634414,-0.215543831721854,-0.848045010612801));
#112799=DIRECTION('center_axis',(-1.4081690688991E-16,0.,-1.));
#112800=DIRECTION('ref_axis',(1.,1.4210854715202E-14,-1.4081690688991E-16));
#112801=DIRECTION('',(0.503989299991708,0.163751169365662,0.848045010612789));
#112802=DIRECTION('center_axis',(-1.4081690688991E-16,0.,-1.));
#112803=DIRECTION('ref_axis',(1.,1.36601840949879E-12,-1.4081690688991E-16));
#112804=DIRECTION('',(-0.503986431075205,-0.163759998982731,-0.848045010612794));
#112805=DIRECTION('center_axis',(-1.4081690688991E-16,0.,-1.));
#112806=DIRECTION('ref_axis',(1.,1.24344978758018E-14,-1.4081690688991E-16));
#112807=DIRECTION('',(0.518345051965145,0.11017289629483,0.848045010612797));
#112808=DIRECTION('center_axis',(-1.4081690688991E-16,0.,-1.));
#112809=DIRECTION('ref_axis',(1.,2.78088663208109E-12,-1.4081690688991E-16));
#112810=DIRECTION('',(-0.518343121711179,-0.110181977425766,-0.848045010612796));
#112811=DIRECTION('center_axis',(-1.4081690688991E-16,0.,-1.));
#112812=DIRECTION('ref_axis',(1.,1.50990331349021E-14,-1.4081690688991E-16));
#112813=DIRECTION('',(0.527021707078575,0.0553875459170368,0.848045010612805));
#112814=DIRECTION('center_axis',(-1.4081690688991E-16,0.,-1.));
#112815=DIRECTION('ref_axis',(1.,2.65121258280487E-12,-1.4081690688991E-16));
#112816=DIRECTION('',(-0.527020736635419,-0.0553967790670736,-0.848045010612794));
#112817=DIRECTION('center_axis',(-1.4081690688991E-16,0.,-1.));
#112818=DIRECTION('ref_axis',(1.,2.8421709430404E-14,-1.4081690688991E-16));
#112819=DIRECTION('',(0.529924202082878,-4.64200440404581E-6,0.848045010612808));
#112820=DIRECTION('center_axis',(-1.4081690688991E-16,0.,-1.));
#112821=DIRECTION('ref_axis',(-1.,0.,1.4081690688991E-16));
#112822=DIRECTION('',(-0.529924689637704,-5.13655126081386E-6,-0.848044705947746));
#112823=DIRECTION('center_axis',(1.4081690688991E-16,0.,1.));
#112824=DIRECTION('ref_axis',(-1.,0.,1.4081690688991E-16));
#112825=DIRECTION('',(0.527022243656738,0.0553871050427197,0.848044705947749));
#112826=DIRECTION('center_axis',(1.4081690688991E-16,0.,1.));
#112827=DIRECTION('ref_axis',(-1.,0.,1.4081690688991E-16));
#112828=DIRECTION('',(-0.527021169825119,-0.0553973218681122,-0.848044705947749));
#112829=DIRECTION('center_axis',(1.4081690688991E-16,0.,1.));
#112830=DIRECTION('ref_axis',(-1.,0.,1.4081690688991E-16));
#112831=DIRECTION('',(0.518345631687774,0.110172513923361,0.848044705947752));
#112832=DIRECTION('center_axis',(1.4081690688991E-16,0.,1.));
#112833=DIRECTION('ref_axis',(-1.,-1.06581410364015E-14,1.4081690688991E-16));
#112834=DIRECTION('',(-0.51834349578966,-0.110182562533937,-0.848044705947753));
#112835=DIRECTION('center_axis',(1.4081690688991E-16,0.,1.));
#112836=DIRECTION('ref_axis',(-1.,0.,1.4081690688991E-16));
#112837=DIRECTION('',(0.503989916507264,0.163750849686365,0.848044705947744));
#112838=DIRECTION('center_axis',(1.4081690688991E-16,0.,1.));
#112839=DIRECTION('ref_axis',(-1.,-3.37507799486048E-14,1.4081690688991E-16));
#112840=DIRECTION('',(-0.503986741943991,-0.163760619987463,-0.848044705947748));
#112841=DIRECTION('center_axis',(1.4081690688991E-16,0.,1.));
#112842=DIRECTION('ref_axis',(-1.,0.,1.4081690688991E-16));
#112843=DIRECTION('',(0.484112382334809,0.215535096873149,0.848044705947745));
#112844=DIRECTION('center_axis',(1.4081690688991E-16,0.,1.));
#112845=DIRECTION('ref_axis',(-1.,4.52970994047064E-14,1.4081690688991E-16));
#112846=DIRECTION('',(-0.484108203887568,-0.215544481819287,-0.848044705947751));
#112847=DIRECTION('center_axis',(1.4081690688991E-16,0.,1.));
#112848=DIRECTION('ref_axis',(-1.,8.88178419700125E-16,1.4081690688991E-16));
#112849=DIRECTION('',(0.458930811594459,0.264957896434965,0.848044705947752));
#112850=DIRECTION('center_axis',(1.4081690688991E-16,0.,1.));
#112851=DIRECTION('ref_axis',(-1.,0.,1.4081690688991E-16));
#112852=DIRECTION('',(-0.458925675043201,-0.264966793202732,-0.848044705947748));
#112853=DIRECTION('center_axis',(1.4081690688991E-16,0.,1.));
#112854=DIRECTION('ref_axis',(-1.,8.88178419700125E-16,1.4081690688991E-16));
#112855=DIRECTION('',(0.428721098844843,0.311477761837432,0.848044705947755));
#112856=DIRECTION('center_axis',(1.4081690688991E-16,0.,1.));
#112857=DIRECTION('ref_axis',(-1.,0.,1.4081690688991E-16));
#112858=DIRECTION('',(-0.428715060466688,-0.311486072951955,-0.848044705947755));
#112859=DIRECTION('center_axis',(1.4081690688991E-16,0.,1.));
#112860=DIRECTION('ref_axis',(-1.,0.,1.4081690688991E-16));
#112861=DIRECTION('',(0.393814228020629,0.35458501170031,0.84804470594775));
#112862=DIRECTION('center_axis',(1.4081690688991E-16,0.,1.));
#112863=DIRECTION('ref_axis',(-1.,1.58095758706622E-13,1.4081690688991E-16));
#112864=DIRECTION('',(-0.393807353973302,-0.354592646103312,-0.848044705947745));
#112865=DIRECTION('center_axis',(1.4081690688991E-16,0.,1.));
#112866=DIRECTION('ref_axis',(-1.,0.,1.4081690688991E-16));
#112867=DIRECTION('',(0.354592646103303,0.393807353973298,0.848044705947751));
#112868=DIRECTION('center_axis',(1.4081690688991E-16,0.,1.));
#112869=DIRECTION('ref_axis',(-1.,0.,1.4081690688991E-16));
#112870=DIRECTION('',(-0.354585011700314,-0.39381422802064,-0.848044705947744));
#112871=DIRECTION('center_axis',(1.4081690688991E-16,0.,1.));
#112872=DIRECTION('ref_axis',(-1.,0.,1.4081690688991E-16));
#112873=DIRECTION('',(0.311486072951974,0.428715060466701,0.848044705947741));
#112874=DIRECTION('center_axis',(1.4081690688991E-16,0.,1.));
#112875=DIRECTION('ref_axis',(-1.,0.,1.4081690688991E-16));
#112876=DIRECTION('',(-0.311477761837448,-0.428721098844851,-0.848044705947745));
#112877=DIRECTION('center_axis',(1.4081690688991E-16,0.,1.));
#112878=DIRECTION('ref_axis',(-1.,0.,1.4081690688991E-16));
#112879=DIRECTION('',(0.264966793202734,0.458925675043206,0.848044705947745));
#112880=DIRECTION('center_axis',(1.4081690688991E-16,0.,1.));
#112881=DIRECTION('ref_axis',(-1.,0.,1.4081690688991E-16));
#112882=DIRECTION('',(-0.264957896434977,-0.458930811594472,-0.848044705947741));
#112883=DIRECTION('center_axis',(1.4081690688991E-16,0.,1.));
#112884=DIRECTION('ref_axis',(-1.,0.,1.4081690688991E-16));
#112885=DIRECTION('',(0.215544481819297,0.484108203887561,0.848044705947752));
#112886=DIRECTION('center_axis',(1.4081690688991E-16,0.,1.));
#112887=DIRECTION('ref_axis',(-1.,0.,1.4081690688991E-16));
#112888=DIRECTION('',(-0.215535096873163,-0.484112382334796,-0.848044705947749));
#112889=DIRECTION('center_axis',(1.4081690688991E-16,0.,1.));
#112890=DIRECTION('ref_axis',(-1.,0.,1.4081690688991E-16));
#112891=DIRECTION('',(0.163760619987462,0.503986741944001,0.848044705947743));
#112892=DIRECTION('center_axis',(1.4081690688991E-16,0.,1.));
#112893=DIRECTION('ref_axis',(-1.,0.,1.4081690688991E-16));
#112894=DIRECTION('',(-0.163750849686385,-0.50398991650724,-0.848044705947753));
#112895=DIRECTION('center_axis',(1.4081690688991E-16,0.,1.));
#112896=DIRECTION('ref_axis',(-1.,0.,1.4081690688991E-16));
#112897=DIRECTION('',(0.11018256253394,0.518343495789649,0.848044705947759));
#112898=DIRECTION('center_axis',(1.4081690688991E-16,0.,1.));
#112899=DIRECTION('ref_axis',(-1.,0.,1.4081690688991E-16));
#112900=DIRECTION('',(-0.110172513923363,-0.51834563168778,-0.848044705947748));
#112901=DIRECTION('center_axis',(1.4081690688991E-16,0.,1.));
#112902=DIRECTION('ref_axis',(-1.,0.,1.4081690688991E-16));
#112903=DIRECTION('',(0.0553973218681129,0.527021169825112,0.848044705947753));
#112904=DIRECTION('center_axis',(1.4081690688991E-16,0.,1.));
#112905=DIRECTION('ref_axis',(-1.,0.,1.4081690688991E-16));
#112906=DIRECTION('',(-0.0553871050427227,-0.527022243656735,-0.848044705947751));
#112907=DIRECTION('center_axis',(1.4081690688991E-16,0.,1.));
#112908=DIRECTION('ref_axis',(-1.,0.,1.4081690688991E-16));
#112909=DIRECTION('',(5.13655126277483E-6,0.529924689637704,0.848044705947746));
#112910=DIRECTION('center_axis',(1.4081690688991E-16,0.,1.));
#112911=DIRECTION('ref_axis',(-1.,0.,1.4081690688991E-16));
#112912=DIRECTION('',(5.13655125885311E-6,-0.529924689637701,-0.848044705947748));
#112913=DIRECTION('center_axis',(1.4081690688991E-16,0.,1.));
#112914=DIRECTION('ref_axis',(-1.,0.,1.4081690688991E-16));
#112915=DIRECTION('',(-0.0553871050427194,0.527022243656735,0.848044705947751));
#112916=DIRECTION('center_axis',(1.4081690688991E-16,0.,1.));
#112917=DIRECTION('ref_axis',(-1.,0.,1.4081690688991E-16));
#112918=DIRECTION('',(0.05539732186811,-0.527021169825103,-0.848044705947759));
#112919=DIRECTION('center_axis',(1.4081690688991E-16,0.,1.));
#112920=DIRECTION('ref_axis',(-1.,0.,1.4081690688991E-16));
#112921=DIRECTION('',(-0.110172513923355,0.518345631687787,0.848044705947745));
#112922=DIRECTION('center_axis',(1.4081690688991E-16,0.,1.));
#112923=DIRECTION('ref_axis',(-1.,0.,1.4081690688991E-16));
#112924=DIRECTION('',(0.110182562533938,-0.518343495789665,-0.848044705947749));
#112925=DIRECTION('center_axis',(1.4081690688991E-16,0.,1.));
#112926=DIRECTION('ref_axis',(-1.,0.,1.4081690688991E-16));
#112927=DIRECTION('',(-0.163750849686367,0.503989916507261,0.848044705947745));
#112928=DIRECTION('center_axis',(1.4081690688991E-16,0.,1.));
#112929=DIRECTION('ref_axis',(-1.,0.,1.4081690688991E-16));
#112930=DIRECTION('',(0.16376061998747,-0.503986741943981,-0.848044705947753));
#112931=DIRECTION('center_axis',(1.4081690688991E-16,0.,1.));
#112932=DIRECTION('ref_axis',(-1.,0.,1.4081690688991E-16));
#112933=DIRECTION('',(-0.215535096873147,0.484112382334806,0.848044705947747));
#112934=DIRECTION('center_axis',(1.4081690688991E-16,0.,1.));
#112935=DIRECTION('ref_axis',(-1.,0.,1.4081690688991E-16));
#112936=DIRECTION('',(0.215544481819295,-0.48410820388757,-0.848044705947748));
#112937=DIRECTION('center_axis',(1.4081690688991E-16,0.,1.));
#112938=DIRECTION('ref_axis',(-1.,5.32907051820075E-15,1.4081690688991E-16));
#112939=DIRECTION('',(-0.264957896434961,0.458930811594451,0.848044705947758));
#112940=DIRECTION('center_axis',(1.4081690688991E-16,0.,1.));
#112941=DIRECTION('ref_axis',(-1.,1.80122583515185E-12,1.4081690688991E-16));
#112942=DIRECTION('',(0.264966793202732,-0.458925675043203,-0.848044705947747));
#112943=DIRECTION('center_axis',(1.4081690688991E-16,0.,1.));
#112944=DIRECTION('ref_axis',(-1.,1.06581410364015E-14,1.4081690688991E-16));
#112945=DIRECTION('',(-0.311477761837441,0.428721098844847,0.84804470594775));
#112946=DIRECTION('center_axis',(1.4081690688991E-16,0.,1.));
#112947=DIRECTION('ref_axis',(-1.,-1.89182003396127E-12,1.4081690688991E-16));
#112948=DIRECTION('',(0.311486072951959,-0.428715060466685,-0.848044705947755));
#112949=DIRECTION('center_axis',(1.4081690688991E-16,0.,1.));
#112950=DIRECTION('ref_axis',(-1.,1.06581410364015E-14,1.4081690688991E-16));
#112951=DIRECTION('',(-0.354585011700304,0.393814228020636,0.84804470594775));
#112952=DIRECTION('center_axis',(1.4081690688991E-16,0.,1.));
#112953=DIRECTION('ref_axis',(-1.,0.,1.4081690688991E-16));
#112954=DIRECTION('',(0.354592646103297,-0.393807353973294,-0.848044705947755));
#112955=DIRECTION('center_axis',(1.4081690688991E-16,0.,1.));
#112956=DIRECTION('ref_axis',(-1.,0.,1.4081690688991E-16));
#112957=DIRECTION('',(-0.393807353973316,0.354592646103293,0.848044705947747));
#112958=DIRECTION('center_axis',(1.4081690688991E-16,0.,1.));
#112959=DIRECTION('ref_axis',(-1.,0.,1.4081690688991E-16));
#112960=DIRECTION('',(0.39381422802063,-0.354585011700304,-0.848044705947752));
#112961=DIRECTION('center_axis',(1.4081690688991E-16,0.,1.));
#112962=DIRECTION('ref_axis',(-1.,0.,1.4081690688991E-16));
#112963=DIRECTION('',(-0.428715060466685,0.311486072951973,0.848044705947749));
#112964=DIRECTION('center_axis',(1.4081690688991E-16,0.,1.));
#112965=DIRECTION('ref_axis',(-1.,2.1618262735501E-12,1.4081690688991E-16));
#112966=DIRECTION('',(0.428721098844842,-0.311477761837438,-0.848044705947753));
#112967=DIRECTION('center_axis',(1.4081690688991E-16,0.,1.));
#112968=DIRECTION('ref_axis',(-1.,0.,1.4081690688991E-16));
#112969=DIRECTION('',(-0.458925675043201,0.264966793202732,0.848044705947748));
#112970=DIRECTION('center_axis',(1.4081690688991E-16,0.,1.));
#112971=DIRECTION('ref_axis',(-1.,-2.25064411552012E-12,1.4081690688991E-16));
#112972=DIRECTION('',(0.458930811594463,-0.264957896434973,-0.848044705947748));
#112973=DIRECTION('center_axis',(1.4081690688991E-16,0.,1.));
#112974=DIRECTION('ref_axis',(-1.,0.,1.4081690688991E-16));
#112975=DIRECTION('',(-0.484108203887567,0.2155444818193,0.848044705947749));
#112976=DIRECTION('center_axis',(1.4081690688991E-16,0.,1.));
#112977=DIRECTION('ref_axis',(-1.,-2.34123831432953E-12,1.4081690688991E-16));
#112978=DIRECTION('',(0.484112382334804,-0.215535096873146,-0.848044705947749));
#112979=DIRECTION('center_axis',(1.4081690688991E-16,0.,1.));
#112980=DIRECTION('ref_axis',(-1.,0.,1.4081690688991E-16));
#112981=DIRECTION('',(-0.503986741943987,0.163760619987466,0.84804470594775));
#112982=DIRECTION('center_axis',(1.4081690688991E-16,0.,1.));
#112983=DIRECTION('ref_axis',(-1.,-2.43183251313894E-12,1.4081690688991E-16));
#112984=DIRECTION('',(0.503989916507253,-0.163750849686376,-0.848044705947748));
#112985=DIRECTION('center_axis',(1.4081690688991E-16,0.,1.));
#112986=DIRECTION('ref_axis',(-1.,0.,1.4081690688991E-16));
#112987=DIRECTION('',(-0.518343495789665,0.110182562533942,0.848044705947749));
#112988=DIRECTION('center_axis',(1.4081690688991E-16,0.,1.));
#112989=DIRECTION('ref_axis',(-1.,-2.52153853352866E-12,1.4081690688991E-16));
#112990=DIRECTION('',(0.518345631687777,-0.110172513923362,-0.84804470594775));
#112991=DIRECTION('center_axis',(1.4081690688991E-16,0.,1.));
#112992=DIRECTION('ref_axis',(-1.,0.,1.4081690688991E-16));
#112993=DIRECTION('',(-0.527021169825119,0.0553973218681105,0.848044705947749));
#112994=DIRECTION('center_axis',(1.4081690688991E-16,0.,1.));
#112995=DIRECTION('ref_axis',(-1.,0.,1.4081690688991E-16));
#112996=DIRECTION('',(0.527022243656741,-0.055387105042722,-0.848044705947747));
#112997=DIRECTION('center_axis',(1.4081690688991E-16,0.,1.));
#112998=DIRECTION('ref_axis',(-1.,0.,1.4081690688991E-16));
#112999=DIRECTION('',(-0.529924689637701,5.13655126091716E-6,0.848044705947748));
#113000=DIRECTION('center_axis',(1.4081690688991E-16,0.,1.));
#113001=DIRECTION('ref_axis',(-1.,0.,1.4081690688991E-16));
#113002=DIRECTION('',(-0.529919264233204,6.48963930749714E-17,0.848048096156427));
#113003=DIRECTION('center_axis',(1.4081690688991E-16,0.,1.));
#113004=DIRECTION('ref_axis',(-1.,0.,1.4081690688991E-16));
#113005=DIRECTION('',(0.529924689637701,5.13655126091716E-6,-0.848044705947748));
#113006=DIRECTION('center_axis',(1.4081690688991E-16,0.,1.));
#113007=DIRECTION('ref_axis',(-1.,0.,1.4081690688991E-16));
#113008=DIRECTION('',(-0.527022243656751,-0.055387105042715,0.848044705947742));
#113009=DIRECTION('center_axis',(1.4081690688991E-16,0.,1.));
#113010=DIRECTION('ref_axis',(-1.,0.,1.4081690688991E-16));
#113011=DIRECTION('',(0.527021169825119,0.0553973218681073,-0.848044705947749));
#113012=DIRECTION('center_axis',(1.4081690688991E-16,0.,1.));
#113013=DIRECTION('ref_axis',(-1.,0.,1.4081690688991E-16));
#113014=DIRECTION('',(-0.518345631687787,-0.110172513923358,0.848044705947744));
#113015=DIRECTION('center_axis',(1.4081690688991E-16,0.,1.));
#113016=DIRECTION('ref_axis',(-1.,0.,1.4081690688991E-16));
#113017=DIRECTION('',(0.518343495789666,0.110182562533928,-0.84804470594775));
#113018=DIRECTION('center_axis',(1.4081690688991E-16,0.,1.));
#113019=DIRECTION('ref_axis',(-1.,0.,1.4081690688991E-16));
#113020=DIRECTION('',(-0.503989916507255,-0.163750849686357,0.848044705947751));
#113021=DIRECTION('center_axis',(1.4081690688991E-16,0.,1.));
#113022=DIRECTION('ref_axis',(-1.,0.,1.4081690688991E-16));
#113023=DIRECTION('',(0.503986741943982,0.163760619987454,-0.848044705947755));
#113024=DIRECTION('center_axis',(1.4081690688991E-16,0.,1.));
#113025=DIRECTION('ref_axis',(-1.,0.,1.4081690688991E-16));
#113026=DIRECTION('',(-0.48411238233481,-0.215535096873142,0.848044705947747));
#113027=DIRECTION('center_axis',(1.4081690688991E-16,0.,1.));
#113028=DIRECTION('ref_axis',(-1.,0.,1.4081690688991E-16));
#113029=DIRECTION('',(0.484108203887574,0.21554448181929,-0.848044705947747));
#113030=DIRECTION('center_axis',(1.4081690688991E-16,0.,1.));
#113031=DIRECTION('ref_axis',(-1.,0.,1.4081690688991E-16));
#113032=DIRECTION('',(-0.458930811594469,-0.264957896434963,0.848044705947747));
#113033=DIRECTION('center_axis',(1.4081690688991E-16,0.,1.));
#113034=DIRECTION('ref_axis',(-1.,0.,1.4081690688991E-16));
#113035=DIRECTION('',(0.458925675043206,0.264966793202728,-0.848044705947747));
#113036=DIRECTION('center_axis',(1.4081690688991E-16,0.,1.));
#113037=DIRECTION('ref_axis',(-1.,0.,1.4081690688991E-16));
#113038=DIRECTION('',(-0.428721098844847,-0.311477761837441,0.84804470594775));
#113039=DIRECTION('center_axis',(1.4081690688991E-16,0.,1.));
#113040=DIRECTION('ref_axis',(-1.,0.,1.4081690688991E-16));
#113041=DIRECTION('',(0.428715060466699,0.311486072951947,-0.848044705947752));
#113042=DIRECTION('center_axis',(1.4081690688991E-16,0.,1.));
#113043=DIRECTION('ref_axis',(-1.,0.,1.4081690688991E-16));
#113044=DIRECTION('',(-0.393814228020627,-0.354585011700295,0.848044705947758));
#113045=DIRECTION('center_axis',(1.4081690688991E-16,0.,1.));
#113046=DIRECTION('ref_axis',(-1.,0.,1.4081690688991E-16));
#113047=DIRECTION('',(0.393807353973304,0.354592646103301,-0.848044705947749));
#113048=DIRECTION('center_axis',(1.4081690688991E-16,0.,1.));
#113049=DIRECTION('ref_axis',(-1.,0.,1.4081690688991E-16));
#113050=DIRECTION('',(-0.354592646103295,-0.393807353973305,0.848044705947751));
#113051=DIRECTION('center_axis',(1.4081690688991E-16,0.,1.));
#113052=DIRECTION('ref_axis',(-1.,0.,1.4081690688991E-16));
#113053=DIRECTION('',(0.354585011700323,0.393814228020616,-0.848044705947751));
#113054=DIRECTION('center_axis',(1.4081690688991E-16,0.,1.));
#113055=DIRECTION('ref_axis',(-1.,0.,1.4081690688991E-16));
#113056=DIRECTION('',(-0.311486072951976,-0.42871506046669,0.848044705947746));
#113057=DIRECTION('center_axis',(1.4081690688991E-16,0.,1.));
#113058=DIRECTION('ref_axis',(-1.,0.,1.4081690688991E-16));
#113059=DIRECTION('',(0.311477761837442,0.428721098844839,-0.848044705947754));
#113060=DIRECTION('center_axis',(1.4081690688991E-16,0.,1.));
#113061=DIRECTION('ref_axis',(-1.,1.95399252334028E-14,1.4081690688991E-16));
#113062=DIRECTION('',(-0.26496679320274,-0.458925675043192,0.848044705947751));
#113063=DIRECTION('center_axis',(1.4081690688991E-16,0.,1.));
#113064=DIRECTION('ref_axis',(-1.,0.,1.4081690688991E-16));
#113065=DIRECTION('',(0.264957896434973,0.458930811594463,-0.848044705947748));
#113066=DIRECTION('center_axis',(1.4081690688991E-16,0.,1.));
#113067=DIRECTION('ref_axis',(-1.,-1.95399252334028E-14,1.4081690688991E-16));
#113068=DIRECTION('',(-0.215544481819302,-0.484108203887559,0.848044705947752));
#113069=DIRECTION('center_axis',(1.4081690688991E-16,0.,1.));
#113070=DIRECTION('ref_axis',(-1.,0.,1.4081690688991E-16));
#113071=DIRECTION('',(0.215535096873159,0.484112382334815,-0.848044705947739));
#113072=DIRECTION('center_axis',(1.4081690688991E-16,0.,1.));
#113073=DIRECTION('ref_axis',(-1.,-9.76996261670138E-15,1.4081690688991E-16));
#113074=DIRECTION('',(-0.163760619987469,-0.503986741944003,0.84804470594774));
#113075=DIRECTION('center_axis',(1.4081690688991E-16,0.,1.));
#113076=DIRECTION('ref_axis',(-1.,-1.89093185554157E-12,1.4081690688991E-16));
#113077=DIRECTION('',(0.163750849686377,0.50398991650726,-0.848044705947744));
#113078=DIRECTION('center_axis',(1.4081690688991E-16,0.,1.));
#113079=DIRECTION('ref_axis',(-1.,-1.06581410364015E-14,1.4081690688991E-16));
#113080=DIRECTION('',(-0.110182562533945,-0.518343495789678,0.848044705947741));
#113081=DIRECTION('center_axis',(1.4081690688991E-16,0.,1.));
#113082=DIRECTION('ref_axis',(-1.,-1.93622895494627E-12,1.4081690688991E-16));
#113083=DIRECTION('',(0.110172513923367,0.51834563168777,-0.848044705947754));
#113084=DIRECTION('center_axis',(1.4081690688991E-16,0.,1.));
#113085=DIRECTION('ref_axis',(-1.,-1.06581410364015E-14,1.4081690688991E-16));
#113086=DIRECTION('',(-0.0553973218681174,-0.527021169825121,0.848044705947747));
#113087=DIRECTION('center_axis',(1.4081690688991E-16,0.,1.));
#113088=DIRECTION('ref_axis',(-1.,-1.98152605435098E-12,1.4081690688991E-16));
#113089=DIRECTION('',(0.0553871050427276,0.527022243656735,-0.848044705947751));
#113090=DIRECTION('center_axis',(1.4081690688991E-16,0.,1.));
#113091=DIRECTION('ref_axis',(-1.,-1.15463194561016E-14,1.4081690688991E-16));
#113092=DIRECTION('',(-5.13655126618051E-6,-0.529924689637704,0.848044705947746));
#113093=DIRECTION('',(-5.13655125534419E-6,0.52992468963771,-0.848044705947742));
#113094=DIRECTION('center_axis',(1.4081690688991E-16,0.,1.));
#113095=DIRECTION('ref_axis',(-1.,-1.15463194561016E-14,1.4081690688991E-16));
#113096=DIRECTION('',(0.0553871050427145,-0.527022243656735,0.848044705947752));
#113097=DIRECTION('center_axis',(1.4081690688991E-16,0.,1.));
#113098=DIRECTION('ref_axis',(-1.,-2.07123207474069E-12,1.4081690688991E-16));
#113099=DIRECTION('',(-0.0553973218681089,0.527021169825119,-0.848044705947749));
#113100=DIRECTION('center_axis',(1.4081690688991E-16,0.,1.));
#113101=DIRECTION('ref_axis',(-1.,-1.15463194561016E-14,1.4081690688991E-16));
#113102=DIRECTION('',(0.110172513923357,-0.518345631687771,0.848044705947754));
#113103=DIRECTION('center_axis',(1.4081690688991E-16,0.,1.));
#113104=DIRECTION('ref_axis',(-1.,-2.1165291741454E-12,1.4081690688991E-16));
#113105=DIRECTION('',(-0.110182562533934,0.518343495789649,-0.848044705947759));
#113106=DIRECTION('center_axis',(1.4081690688991E-16,0.,1.));
#113107=DIRECTION('ref_axis',(-1.,-1.15463194561016E-14,1.4081690688991E-16));
#113108=DIRECTION('',(0.163750849686358,-0.503989916507253,0.848044705947751));
#113109=DIRECTION('center_axis',(1.4081690688991E-16,0.,1.));
#113110=DIRECTION('ref_axis',(-1.,-4.32276436868051E-12,1.4081690688991E-16));
#113111=DIRECTION('',(-0.163760619987469,0.50398674194399,-0.848044705947747));
#113112=DIRECTION('center_axis',(1.4081690688991E-16,0.,1.));
#113113=DIRECTION('ref_axis',(-1.,-1.15463194561016E-14,1.4081690688991E-16));
#113114=DIRECTION('',(0.21553509687315,-0.484112382334798,0.848044705947752));
#113115=DIRECTION('center_axis',(1.4081690688991E-16,0.,1.));
#113116=DIRECTION('ref_axis',(-1.,-2.20623519453511E-12,1.4081690688991E-16));
#113117=DIRECTION('',(-0.215544481819284,0.484108203887573,-0.848044705947749));
#113118=DIRECTION('center_axis',(1.4081690688991E-16,0.,1.));
#113119=DIRECTION('ref_axis',(-1.,-1.24344978758018E-14,1.4081690688991E-16));
#113120=DIRECTION('',(0.264957896434973,-0.458930811594463,0.848044705947748));
#113121=DIRECTION('center_axis',(1.4081690688991E-16,0.,1.));
#113122=DIRECTION('ref_axis',(-1.,-4.50306458787963E-12,1.4081690688991E-16));
#113123=DIRECTION('',(-0.264966793202732,0.458925675043201,-0.848044705947748));
#113124=DIRECTION('center_axis',(1.4081690688991E-16,0.,1.));
#113125=DIRECTION('ref_axis',(-1.,-1.24344978758018E-14,1.4081690688991E-16));
#113126=DIRECTION('',(0.31147776183743,-0.428721098844854,0.84804470594775));
#113127=DIRECTION('center_axis',(1.4081690688991E-16,0.,1.));
#113128=DIRECTION('ref_axis',(-1.,-2.29682939334452E-12,1.4081690688991E-16));
#113129=DIRECTION('',(-0.31148607295195,0.428715060466704,-0.848044705947748));
#113130=DIRECTION('center_axis',(1.4081690688991E-16,0.,1.));
#113131=DIRECTION('ref_axis',(-1.,-3.19744231092045E-14,1.4081690688991E-16));
#113132=DIRECTION('',(0.354585011700312,-0.393814228020624,0.848044705947752));
#113133=DIRECTION('center_axis',(1.4081690688991E-16,0.,1.));
#113134=DIRECTION('ref_axis',(-1.,7.02460312140829E-12,1.4081690688991E-16));
#113135=DIRECTION('',(-0.354592646103303,0.393807353973293,-0.848044705947754));
#113136=DIRECTION('center_axis',(1.4081690688991E-16,0.,1.));
#113137=DIRECTION('ref_axis',(-1.,0.,1.4081690688991E-16));
#113138=DIRECTION('',(0.393807353973315,-0.354592646103299,0.848044705947745));
#113139=DIRECTION('center_axis',(1.4081690688991E-16,0.,1.));
#113140=DIRECTION('ref_axis',(-1.,-1.19282361765727E-12,1.4081690688991E-16));
#113141=DIRECTION('',(-0.393814228020623,0.354585011700318,-0.84804470594775));
#113142=DIRECTION('center_axis',(1.4081690688991E-16,0.,1.));
#113143=DIRECTION('ref_axis',(-1.,-3.28626015289046E-14,1.4081690688991E-16));
#113144=DIRECTION('',(0.428715060466675,-0.311486072951968,0.848044705947756));
#113145=DIRECTION('center_axis',(1.4081690688991E-16,0.,1.));
#113146=DIRECTION('ref_axis',(-1.,-1.21591625656947E-12,1.4081690688991E-16));
#113147=DIRECTION('',(-0.428721098844844,0.311477761837459,-0.848044705947745));
#113148=DIRECTION('center_axis',(1.4081690688991E-16,0.,1.));
#113149=DIRECTION('ref_axis',(-1.,7.105427357601E-15,1.4081690688991E-16));
#113150=DIRECTION('',(0.458925675043201,-0.264966793202732,0.848044705947748));
#113151=DIRECTION('center_axis',(1.4081690688991E-16,0.,1.));
#113152=DIRECTION('ref_axis',(-1.,-4.9533710466676E-12,1.4081690688991E-16));
#113153=DIRECTION('',(-0.458930811594453,0.264957896434968,-0.848044705947754));
#113154=DIRECTION('center_axis',(1.4081690688991E-16,0.,1.));
#113155=DIRECTION('ref_axis',(-1.,-1.33226762955019E-14,1.4081690688991E-16));
#113156=DIRECTION('',(0.484108203887561,-0.21554448181931,0.848044705947749));
#113157=DIRECTION('center_axis',(1.4081690688991E-16,0.,1.));
#113158=DIRECTION('ref_axis',(-1.,-2.52153853352866E-12,1.4081690688991E-16));
#113159=DIRECTION('',(-0.484112382334809,0.215535096873149,-0.848044705947745));
#113160=DIRECTION('center_axis',(1.4081690688991E-16,0.,1.));
#113161=DIRECTION('ref_axis',(-1.,-4.79616346638068E-14,1.4081690688991E-16));
#113162=DIRECTION('',(0.503986741943987,-0.163760619987463,0.848044705947751));
#113163=DIRECTION('center_axis',(1.4081690688991E-16,0.,1.));
#113164=DIRECTION('ref_axis',(-1.,7.70050689880008E-12,1.4081690688991E-16));
#113165=DIRECTION('',(-0.503989916507244,0.163750849686371,-0.848044705947754));
#113166=DIRECTION('center_axis',(1.4081690688991E-16,0.,1.));
#113167=DIRECTION('ref_axis',(-1.,7.105427357601E-15,1.4081690688991E-16));
#113168=DIRECTION('',(0.518343495789671,-0.110182562533949,0.848044705947744));
#113169=DIRECTION('center_axis',(1.4081690688991E-16,0.,1.));
#113170=DIRECTION('ref_axis',(-1.,-2.28528307388842E-12,1.4081690688991E-16));
#113171=DIRECTION('',(-0.518345631687771,0.110172513923364,-0.848044705947753));
#113172=DIRECTION('center_axis',(1.4081690688991E-16,0.,1.));
#113173=DIRECTION('ref_axis',(-1.,1.33226762955019E-14,1.4081690688991E-16));
#113174=DIRECTION('',(0.527021169825115,-0.0553973218681165,0.848044705947751));
#113175=DIRECTION('center_axis',(1.4081690688991E-16,0.,1.));
#113176=DIRECTION('ref_axis',(-1.,-2.65654165332307E-12,1.4081690688991E-16));
#113177=DIRECTION('',(-0.527022243656726,0.0553871050427283,-0.848044705947756));
#113178=DIRECTION('center_axis',(1.4081690688991E-16,0.,1.));
#113179=DIRECTION('ref_axis',(-1.,5.32907051820075E-15,1.4081690688991E-16));
#113180=DIRECTION('',(0.529924689637697,-5.13655126081405E-6,0.84804470594775));
#113181=DIRECTION('center_axis',(1.4081690688991E-16,0.,1.));
#113182=DIRECTION('ref_axis',(1.,0.,-1.4081690688991E-16));
#113183=DIRECTION('center_axis',(-1.4081690688991E-16,0.,-1.));
#113184=DIRECTION('ref_axis',(-1.,0.,1.4081690688991E-16));
#113185=DIRECTION('',(-0.529919264233204,-6.48963930749714E-17,0.848048096156427));
#113186=DIRECTION('center_axis',(-1.4081690688991E-16,0.,-1.));
#113187=DIRECTION('ref_axis',(-1.,0.,1.4081690688991E-16));
#113188=DIRECTION('center_axis',(-1.4081690688991E-16,0.,-1.));
#113189=DIRECTION('ref_axis',(-1.,0.,1.4081690688991E-16));
#113190=DIRECTION('',(-1.40816906889911E-16,0.,-1.));
#113191=DIRECTION('center_axis',(-1.4081690688991E-16,0.,-1.));
#113192=DIRECTION('ref_axis',(-1.,0.,1.4081690688991E-16));
#113193=DIRECTION('center_axis',(-1.4081690688991E-16,0.,-1.));
#113194=DIRECTION('ref_axis',(-1.,0.,1.40816906889911E-16));
#113195=DIRECTION('center_axis',(-1.4081690688991E-16,0.,-1.));
#113196=DIRECTION('ref_axis',(-1.,0.,1.4081690688991E-16));
#113197=DIRECTION('',(-0.994521895368275,-0.10452846326764,1.40045497140052E-16));
#113198=DIRECTION('center_axis',(-1.4081690688991E-16,0.,-1.));
#113199=DIRECTION('ref_axis',(-1.,0.,1.4081690688991E-16));
#113200=DIRECTION('',(1.,0.,-1.40816906889911E-16));
#113201=DIRECTION('center_axis',(-1.4081690688991E-16,0.,-1.));
#113202=DIRECTION('ref_axis',(-1.,0.,1.4081690688991E-16));
#113203=DIRECTION('center_axis',(-1.4081690688991E-16,0.,-1.));
#113204=DIRECTION('ref_axis',(-1.,0.,1.4081690688991E-16));
#113205=DIRECTION('center_axis',(1.4081690688991E-16,0.,1.));
#113206=DIRECTION('ref_axis',(1.,0.,-1.4081690688991E-16));
#113207=DIRECTION('center_axis',(1.4081690688991E-16,0.,1.));
#113208=DIRECTION('ref_axis',(-1.,0.,1.40816906889911E-16));
#113209=DIRECTION('',(-0.4972656110608,-0.0522695260941939,-0.866022406579771));
#113210=DIRECTION('',(0.500005191251964,-4.7780011657308E-6,0.866022406579794));
#113211=DIRECTION('center_axis',(-1.4081690688991E-16,0.,-1.));
#113212=DIRECTION('ref_axis',(-1.,0.,1.40816906889911E-16));
#113213=DIRECTION('center_axis',(1.4081690688991E-16,0.,1.));
#113214=DIRECTION('ref_axis',(-1.,0.,1.4081690688991E-16));
#113215=DIRECTION('',(-0.994521895368275,-0.10452846326764,1.40045497140052E-16));
#113216=DIRECTION('center_axis',(-1.4081690688991E-16,0.,-1.));
#113217=DIRECTION('ref_axis',(-1.,0.,1.4081690688991E-16));
#113218=DIRECTION('',(1.,0.,-1.40816906889911E-16));
#113219=DIRECTION('center_axis',(-1.4081690688991E-16,0.,-1.));
#113220=DIRECTION('ref_axis',(-1.,0.,1.4081690688991E-16));
#113221=DIRECTION('center_axis',(-1.4081690688991E-16,0.,-1.));
#113222=DIRECTION('ref_axis',(-1.,0.,1.4081690688991E-16));
#113223=DIRECTION('',(-0.497266395846506,-0.052260151065429,0.86602252174666));
#113224=DIRECTION('center_axis',(-1.4081690688991E-16,0.,-1.));
#113225=DIRECTION('ref_axis',(1.,3.46389583683049E-14,-1.4081690688991E-16));
#113226=DIRECTION('',(0.500004991781248,4.62770265276801E-6,-0.866022521746645));
#113227=DIRECTION('center_axis',(-1.4081690688991E-16,0.,-1.));
#113228=DIRECTION('ref_axis',(-1.,0.,1.4081690688991E-16));
#113229=DIRECTION('center_axis',(-1.4081690688991E-16,0.,-1.));
#113230=DIRECTION('ref_axis',(-1.,0.,1.4081690688991E-16));
#113231=DIRECTION('center_axis',(-1.4081690688991E-16,0.,-1.));
#113232=DIRECTION('ref_axis',(-1.,0.,1.40816906889911E-16));
#113233=DIRECTION('center_axis',(1.4081690688991E-16,0.,1.));
#113234=DIRECTION('ref_axis',(-1.,0.,1.4081690688991E-16));
#113235=DIRECTION('',(-0.994521895368275,-0.10452846326764,1.40045497140052E-16));
#113236=DIRECTION('',(1.,0.,-1.40816906889911E-16));
#113237=DIRECTION('center_axis',(-1.4081690688991E-16,0.,-1.));
#113238=DIRECTION('ref_axis',(-1.,0.,1.17174841180864E-16));
#113239=DIRECTION('center_axis',(-0.103464010407628,0.994633197962203,7.86457232110799E-6));
#113240=DIRECTION('ref_axis',(-0.843493966781864,-0.0877379732620273,-0.529924500330441));
#113241=DIRECTION('center_axis',(0.00107025596476198,-0.999999427244995,
7.86457194324946E-6));
#113242=DIRECTION('ref_axis',(1.47312952164193E-6,-7.86299982088955E-6,
-0.999999999968001));
#113243=DIRECTION('center_axis',(-1.4081690688991E-16,0.,-1.));
#113244=DIRECTION('ref_axis',(-1.,0.,1.13676889660403E-16));
#113245=DIRECTION('center_axis',(-0.103509373496897,0.994628478127797,-9.77051512295647E-6));
#113246=DIRECTION('ref_axis',(0.869950553189208,0.0905391058403171,0.48475633602814));
#113247=DIRECTION('center_axis',(0.00102464806165023,-0.999999475000305,
-9.77058602570879E-6));
#113248=DIRECTION('ref_axis',(0.874641264345339,0.000891463458077043,0.484769908304229));
#113249=DIRECTION('center_axis',(-1.4081690688991E-16,0.,-1.));
#113250=DIRECTION('ref_axis',(-1.,0.,1.15974593313694E-16));
#113251=DIRECTION('center_axis',(0.107112171226392,-0.994246942387258,1.81316452328514E-5));
#113252=DIRECTION('ref_axis',(0.861994650487305,0.0928552846708997,-0.498340364249129));
#113253=DIRECTION('center_axis',(0.0025983123505628,0.999996624215829,1.81624797792123E-5));
#113254=DIRECTION('ref_axis',(0.865241946196498,-0.0022390706427668,-0.501349539846954));
#113255=DIRECTION('center_axis',(-1.4081690688991E-16,0.,-1.));
#113256=DIRECTION('ref_axis',(-1.,0.,1.16261524579732E-16));
#113257=DIRECTION('center_axis',(0.10712560498394,-0.994245495043162,1.85257085273757E-5));
#113258=DIRECTION('ref_axis',(0.860265387812352,0.0926991758191971,0.501348506863744));
#113259=DIRECTION('center_axis',(0.00261182427506424,0.999996589010146,
1.84940601154894E-5));
#113260=DIRECTION('ref_axis',(0.866979057021487,-0.00227362102099331,0.498339387700376));
#113261=DIRECTION('center_axis',(-1.4081690688991E-16,0.,-1.));
#113262=DIRECTION('ref_axis',(-1.,0.,1.40816906889911E-16));
#113263=DIRECTION('center_axis',(-1.4081690688991E-16,0.,-1.));
#113264=DIRECTION('ref_axis',(-1.,0.,1.4081690688991E-16));
#113265=DIRECTION('',(0.994521895368275,0.10452846326764,-1.40045497140052E-16));
#113266=DIRECTION('center_axis',(-1.4081690688991E-16,0.,-1.));
#113267=DIRECTION('ref_axis',(-1.,0.,1.4081690688991E-16));
#113268=DIRECTION('center_axis',(-1.4081690688991E-16,0.,-1.));
#113269=DIRECTION('ref_axis',(-1.,0.,1.4081690688991E-16));
#113270=DIRECTION('center_axis',(-1.4081690688991E-16,0.,-1.));
#113271=DIRECTION('ref_axis',(-1.,0.,1.4081690688991E-16));
#113272=DIRECTION('',(-0.978147600733808,-0.207911690817747,1.37739719617122E-16));
#113273=DIRECTION('center_axis',(1.4081690688991E-16,0.,1.));
#113274=DIRECTION('ref_axis',(1.,0.,-1.4081690688991E-16));
#113275=DIRECTION('',(0.497266609935015,0.0522600224406397,0.866022406579784));
#113276=DIRECTION('center_axis',(1.4081690688991E-16,0.,1.));
#113277=DIRECTION('ref_axis',(-1.,0.,1.40816906889911E-16));
#113278=DIRECTION('',(-0.489077884775286,-0.103961598321231,-0.866022406579776));
#113279=DIRECTION('center_axis',(-1.4081690688991E-16,0.,-1.));
#113280=DIRECTION('ref_axis',(-1.,0.,1.40816906889911E-16));
#113281=DIRECTION('center_axis',(-1.4081690688991E-16,0.,-1.));
#113282=DIRECTION('ref_axis',(-1.,0.,1.4081690688991E-16));
#113283=DIRECTION('',(0.994521895368275,0.10452846326764,-1.40045497140052E-16));
#113284=DIRECTION('center_axis',(1.4081690688991E-16,0.,1.));
#113285=DIRECTION('ref_axis',(-1.,0.,1.4081690688991E-16));
#113286=DIRECTION('',(-0.978147600733808,-0.207911690817747,1.37739719617122E-16));
#113287=DIRECTION('center_axis',(-1.4081690688991E-16,0.,-1.));
#113288=DIRECTION('ref_axis',(-1.,0.,1.4081690688991E-16));
#113289=DIRECTION('center_axis',(-1.4081690688991E-16,0.,-1.));
#113290=DIRECTION('ref_axis',(1.,1.86517468137026E-14,-1.4081690688991E-16));
#113291=DIRECTION('',(0.497265428393217,0.0522693557686574,-0.866022521746658));
#113292=DIRECTION('center_axis',(-1.4081690688991E-16,0.,-1.));
#113293=DIRECTION('ref_axis',(-1.,0.,1.4081690688991E-16));
#113294=DIRECTION('center_axis',(-1.4081690688991E-16,0.,-1.));
#113295=DIRECTION('ref_axis',(-1.,0.,1.4081690688991E-16));
#113296=DIRECTION('center_axis',(-1.4081690688991E-16,0.,-1.));
#113297=DIRECTION('ref_axis',(-1.,0.,1.4081690688991E-16));
#113298=DIRECTION('',(-0.489079645219225,-0.1039523566823,0.866022521746653));
#113299=DIRECTION('center_axis',(-1.4081690688991E-16,0.,-1.));
#113300=DIRECTION('ref_axis',(-1.,0.,1.40816906889911E-16));
#113301=DIRECTION('',(0.994521895368275,0.10452846326764,-1.40045497140052E-16));
#113302=DIRECTION('center_axis',(1.4081690688991E-16,0.,1.));
#113303=DIRECTION('ref_axis',(-1.,0.,1.4081690688991E-16));
#113304=DIRECTION('',(-0.978147600733808,-0.207911690817747,1.37739719617122E-16));
#113305=DIRECTION('center_axis',(-1.4081690688991E-16,0.,-1.));
#113306=DIRECTION('ref_axis',(-1.,0.,1.17174841180864E-16));
#113307=DIRECTION('center_axis',(0.105592796389087,-0.994409453539578,7.8645721102773E-6));
#113308=DIRECTION('ref_axis',(2.28696687445886E-6,-7.66594168623456E-6,
-0.999999999968001));
#113309=DIRECTION('center_axis',(-0.206864703431098,0.978369559222134,7.86457219200017E-6));
#113310=DIRECTION('ref_axis',(-0.829702103060253,-0.175426463587734,-0.529924500330466));
#113311=DIRECTION('center_axis',(-1.4081690688991E-16,0.,-1.));
#113312=DIRECTION('ref_axis',(-1.,0.,1.13676889660403E-16));
#113313=DIRECTION('center_axis',(0.105547443322395,-0.994414268357329,-9.7705855822117E-6));
#113314=DIRECTION('ref_axis',(0.869756704680254,0.0923114872006744,0.484769908301397));
#113315=DIRECTION('center_axis',(-0.206909324659144,0.978360123509556,-9.77051573642606E-6));
#113316=DIRECTION('ref_axis',(0.855720959435962,0.18097771758913,0.484756336026901));
#113317=DIRECTION('center_axis',(-1.4081690688991E-16,0.,-1.));
#113318=DIRECTION('ref_axis',(-1.,0.,1.15974593313694E-16));
#113319=DIRECTION('center_axis',(-0.101944031878512,0.994790135674091,1.81624797640825E-5));
#113320=DIRECTION('ref_axis',(0.860736106896466,0.0882156062110998,-0.501349539847723));
#113321=DIRECTION('center_axis',(0.210452504541384,-0.97760408295153,1.81316452299207E-5));
#113322=DIRECTION('ref_axis',(0.847566533387361,0.182449589866313,-0.498340364248519));
#113323=DIRECTION('center_axis',(-1.4081690688991E-16,0.,-1.));
#113324=DIRECTION('ref_axis',(-1.,0.,1.16261524579732E-16));
#113325=DIRECTION('center_axis',(-0.101930590293366,0.994791513042012,1.84940595419896E-5));
#113326=DIRECTION('ref_axis',(0.862467313148182,0.0883628226288529,0.498339387694789));
#113327=DIRECTION('center_axis',(0.210465713413753,-0.97760123932718,1.85257174127305E-5));
#113328=DIRECTION('ref_axis',(0.845863061616564,0.182113579026111,0.501348506856213));
#113329=DIRECTION('center_axis',(-1.4081690688991E-16,0.,-1.));
#113330=DIRECTION('ref_axis',(-1.,0.,1.40816906889911E-16));
#113331=DIRECTION('center_axis',(-1.4081690688991E-16,0.,-1.));
#113332=DIRECTION('ref_axis',(-1.,0.,1.4081690688991E-16));
#113333=DIRECTION('',(0.978147600733808,0.207911690817747,-1.37739719617122E-16));
#113334=DIRECTION('center_axis',(-1.4081690688991E-16,0.,-1.));
#113335=DIRECTION('ref_axis',(-1.,0.,1.4081690688991E-16));
#113336=DIRECTION('center_axis',(-1.4081690688991E-16,0.,-1.));
#113337=DIRECTION('ref_axis',(-1.,0.,1.4081690688991E-16));
#113338=DIRECTION('center_axis',(-1.4081690688991E-16,0.,-1.));
#113339=DIRECTION('ref_axis',(-1.,0.,1.4081690688991E-16));
#113340=DIRECTION('',(-0.951056516295158,-0.309016994374935,1.33924836902178E-16));
#113341=DIRECTION('center_axis',(1.4081690688991E-16,0.,1.));
#113342=DIRECTION('ref_axis',(1.,0.,-1.4081690688991E-16));
#113343=DIRECTION('',(0.489079871579873,0.103952251140473,0.866022406579786));
#113344=DIRECTION('center_axis',(1.4081690688991E-16,0.,1.));
#113345=DIRECTION('ref_axis',(-1.,0.,1.40816906889911E-16));
#113346=DIRECTION('',(-0.475531718838024,-0.154514645521702,-0.866022406579793));
#113347=DIRECTION('center_axis',(-1.4081690688991E-16,0.,-1.));
#113348=DIRECTION('ref_axis',(-1.,0.,1.40816906889911E-16));
#113349=DIRECTION('center_axis',(-1.4081690688991E-16,0.,-1.));
#113350=DIRECTION('ref_axis',(-1.,0.,1.4081690688991E-16));
#113351=DIRECTION('',(0.978147600733808,0.207911690817747,-1.37739719617122E-16));
#113352=DIRECTION('center_axis',(1.4081690688991E-16,0.,1.));
#113353=DIRECTION('ref_axis',(-1.,0.,1.4081690688991E-16));
#113354=DIRECTION('',(-0.951056516295158,-0.309016994374935,1.33924836902178E-16));
#113355=DIRECTION('center_axis',(-1.4081690688991E-16,0.,-1.));
#113356=DIRECTION('ref_axis',(-1.,0.,1.4081690688991E-16));
#113357=DIRECTION('center_axis',(-1.4081690688991E-16,0.,-1.));
#113358=DIRECTION('ref_axis',(1.,1.4210854715202E-14,-1.4081690688991E-16));
#113359=DIRECTION('',(0.489077720912263,0.103961409834796,-0.866022521746651));
#113360=DIRECTION('center_axis',(-1.4081690688991E-16,0.,-1.));
#113361=DIRECTION('ref_axis',(-1.,0.,1.4081690688991E-16));
#113362=DIRECTION('center_axis',(-1.4081690688991E-16,0.,-1.));
#113363=DIRECTION('ref_axis',(-1.,0.,1.4081690688991E-16));
#113364=DIRECTION('center_axis',(-1.4081690688991E-16,0.,-1.));
#113365=DIRECTION('ref_axis',(-1.,0.,1.4081690688991E-16));
#113366=DIRECTION('',(-0.475534435652402,-0.154505638525938,0.86602252174666));
#113367=DIRECTION('center_axis',(-1.4081690688991E-16,0.,-1.));
#113368=DIRECTION('ref_axis',(-1.,0.,1.40816906889911E-16));
#113369=DIRECTION('',(0.978147600733808,0.207911690817747,-1.37739719617122E-16));
#113370=DIRECTION('center_axis',(1.4081690688991E-16,0.,1.));
#113371=DIRECTION('ref_axis',(-1.,0.,1.4081690688991E-16));
#113372=DIRECTION('',(-0.951056516295158,-0.309016994374935,1.33924836902178E-16));
#113373=DIRECTION('center_axis',(-1.4081690688991E-16,0.,-1.));
#113374=DIRECTION('ref_axis',(-1.,0.,1.17174841180864E-16));
#113375=DIRECTION('center_axis',(0.208958440039433,-0.977924521767624,7.86457212166731E-6));
#113376=DIRECTION('ref_axis',(3.07574774830936E-6,-7.38489373063671E-6,
-0.999999999968002));
#113377=DIRECTION('center_axis',(-0.307998943474316,0.951386698854285,7.86457231463923E-6));
#113378=DIRECTION('ref_axis',(-0.806819849471271,-0.261192944867695,-0.529924500330468));
#113379=DIRECTION('center_axis',(-1.4081690688991E-16,0.,-1.));
#113380=DIRECTION('ref_axis',(-1.,0.,1.13676889660403E-16));
#113381=DIRECTION('center_axis',(0.208913838707158,-0.97793405089565,-9.77058570875104E-6));
#113382=DIRECTION('ref_axis',(0.855342908547131,0.182720126971686,0.484769908304533));
#113383=DIRECTION('center_axis',(-0.308042333962507,0.95137265064299,-9.77051511559201E-6));
#113384=DIRECTION('ref_axis',(0.832115907779592,0.269433499592006,0.48475633602641));
#113385=DIRECTION('center_axis',(-1.4081690688991E-16,0.,-1.));
#113386=DIRECTION('ref_axis',(-1.,0.,1.15974593313694E-16));
#113387=DIRECTION('center_axis',(-0.205369455961159,0.978684518232685,1.81624797493655E-5));
#113388=DIRECTION('ref_axis',(0.846799862694007,0.177703774424036,-0.501349539839084));
#113389=DIRECTION('center_axis',(0.31148707617651,-0.95025038860621,1.81316451190475E-5));
#113390=DIRECTION('ref_axis',(0.82385229998115,0.270044939174584,-0.498340364251145));
#113391=DIRECTION('center_axis',(-1.4081690688991E-16,0.,-1.));
#113392=DIRECTION('ref_axis',(-1.,0.,1.16261524579732E-16));
#113393=DIRECTION('center_axis',(-0.205356231984476,0.9786872930835,1.84940593962113E-5));
#113394=DIRECTION('ref_axis',(0.848506196906012,0.178031144702923,0.498339387694635));
#113395=DIRECTION('center_axis',(0.311499915448403,-0.950246179856797,1.8525719752645E-5));
#113396=DIRECTION('ref_axis',(0.822193282702067,0.269532707749979,0.501348506861807));
#113397=DIRECTION('center_axis',(-1.4081690688991E-16,0.,-1.));
#113398=DIRECTION('ref_axis',(-1.,0.,1.40816906889911E-16));
#113399=DIRECTION('center_axis',(-1.4081690688991E-16,0.,-1.));
#113400=DIRECTION('ref_axis',(-1.,0.,1.4081690688991E-16));
#113401=DIRECTION('',(0.951056516295158,0.309016994374935,-1.33924836902178E-16));
#113402=DIRECTION('center_axis',(-1.4081690688991E-16,0.,-1.));
#113403=DIRECTION('ref_axis',(-1.,0.,1.4081690688991E-16));
#113404=DIRECTION('center_axis',(-1.4081690688991E-16,0.,-1.));
#113405=DIRECTION('ref_axis',(-1.,0.,1.4081690688991E-16));
#113406=DIRECTION('center_axis',(-1.4081690688991E-16,0.,-1.));
#113407=DIRECTION('ref_axis',(-1.,0.,1.4081690688991E-16));
#113408=DIRECTION('',(-0.913545457642606,-0.406736643075789,1.2864264564856E-16));
#113409=DIRECTION('center_axis',(1.4081690688991E-16,0.,1.));
#113410=DIRECTION('ref_axis',(1.,0.,-1.4081690688991E-16));
#113411=DIRECTION('',(0.475534671805143,0.15450555722339,0.866022406579798));
#113412=DIRECTION('center_axis',(1.4081690688991E-16,0.,1.));
#113413=DIRECTION('ref_axis',(-1.,0.,1.40816906889911E-16));
#113414=DIRECTION('',(-0.456775527877824,-0.203374797931539,-0.866022406579784));
#113415=DIRECTION('center_axis',(-1.4081690688991E-16,0.,-1.));
#113416=DIRECTION('ref_axis',(-1.,0.,1.40816906889911E-16));
#113417=DIRECTION('center_axis',(-1.4081690688991E-16,0.,-1.));
#113418=DIRECTION('ref_axis',(-1.,0.,1.4081690688991E-16));
#113419=DIRECTION('',(0.951056516295158,0.309016994374935,-1.33924836902178E-16));
#113420=DIRECTION('center_axis',(1.4081690688991E-16,0.,1.));
#113421=DIRECTION('ref_axis',(-1.,0.,1.4081690688991E-16));
#113422=DIRECTION('',(-0.913545457642606,-0.406736643075789,1.2864264564856E-16));
#113423=DIRECTION('center_axis',(-1.4081690688991E-16,0.,-1.));
#113424=DIRECTION('ref_axis',(-1.,0.,1.4081690688991E-16));
#113425=DIRECTION('center_axis',(-1.4081690688991E-16,0.,-1.));
#113426=DIRECTION('ref_axis',(1.,2.04281036531029E-14,-1.4081690688991E-16));
#113427=DIRECTION('',(0.47553157557488,0.154514440939486,-0.866022521746652));
#113428=DIRECTION('center_axis',(-1.4081690688991E-16,0.,-1.));
#113429=DIRECTION('ref_axis',(-1.,0.,1.4081690688991E-16));
#113430=DIRECTION('center_axis',(-1.4081690688991E-16,0.,-1.));
#113431=DIRECTION('ref_axis',(-1.,0.,1.4081690688991E-16));
#113432=DIRECTION('center_axis',(-1.4081690688991E-16,0.,-1.));
#113433=DIRECTION('ref_axis',(-1.,0.,1.4081690688991E-16));
#113434=DIRECTION('',(-0.456779171296623,-0.203366124261482,0.866022521746654));
#113435=DIRECTION('center_axis',(-1.4081690688991E-16,0.,-1.));
#113436=DIRECTION('ref_axis',(-1.,0.,1.40816906889911E-16));
#113437=DIRECTION('',(0.951056516295158,0.309016994374935,-1.33924836902178E-16));
#113438=DIRECTION('center_axis',(1.4081690688991E-16,0.,1.));
#113439=DIRECTION('ref_axis',(-1.,0.,1.4081690688991E-16));
#113440=DIRECTION('',(-0.913545457642606,-0.406736643075789,1.2864264564856E-16));
#113441=DIRECTION('center_axis',(-1.4081690688991E-16,0.,-1.));
#113442=DIRECTION('ref_axis',(-1.,0.,1.17174841180864E-16));
#113443=DIRECTION('center_axis',(0.310034691293352,-0.950725244291317,7.86457213372142E-6));
#113444=DIRECTION('ref_axis',(3.83083005362731E-6,-7.02293534441516E-6,
-0.999999999968002));
#113445=DIRECTION('center_axis',(-0.405758682640018,0.913980246723301,7.86457234792495E-6));
#113446=DIRECTION('ref_axis',(-0.775097908773559,-0.344097741585692,-0.529924500330455));
#113447=DIRECTION('center_axis',(-1.4081690688991E-16,0.,-1.));
#113448=DIRECTION('ref_axis',(-1.,0.,1.13676889660403E-16));
#113449=DIRECTION('center_axis',(0.309991330356933,-0.950739383326511,-9.77058570930425E-6));
#113450=DIRECTION('ref_axis',(0.831557796517394,0.27112684679503,0.484769908305085));
#113451=DIRECTION('center_axis',(-0.405800366992815,0.913961739928447,-9.77051475421558E-6));
#113452=DIRECTION('ref_axis',(0.799394020106877,0.354937311791151,0.484756336024438));
#113453=DIRECTION('center_axis',(-1.4081690688991E-16,0.,-1.));
#113454=DIRECTION('ref_axis',(-1.,0.,1.15974593313694E-16));
#113455=DIRECTION('center_axis',(-0.306544809307878,0.951856228406644,1.81624797541284E-5));
#113456=DIRECTION('ref_axis',(0.823585901985486,0.265244982896519,-0.501349539841196));
#113457=DIRECTION('center_axis',(0.409108930222434,-0.912485552150553,1.81316453160849E-5));
#113458=DIRECTION('ref_axis',(0.791111768373129,0.354681619617994,-0.498340364255894));
#113459=DIRECTION('center_axis',(-1.4081690688991E-16,0.,-1.));
#113460=DIRECTION('ref_axis',(-1.,0.,1.16261524579732E-16));
#113461=DIRECTION('center_axis',(-0.306531947828759,0.951860370337098,1.84940671411514E-5));
#113462=DIRECTION('ref_axis',(0.825248669203561,0.265748920298447,0.498339387704766));
#113463=DIRECTION('center_axis',(0.409121259222939,-0.912480024388827,1.85257240494735E-5));
#113464=DIRECTION('ref_axis',(0.789515382129665,0.353998779724754,0.501348506863274));
#113465=DIRECTION('center_axis',(-1.4081690688991E-16,0.,-1.));
#113466=DIRECTION('ref_axis',(-1.,0.,1.40816906889911E-16));
#113467=DIRECTION('center_axis',(-1.4081690688991E-16,0.,-1.));
#113468=DIRECTION('ref_axis',(-1.,0.,1.4081690688991E-16));
#113469=DIRECTION('',(0.913545457642606,0.406736643075789,-1.2864264564856E-16));
#113470=DIRECTION('center_axis',(-1.4081690688991E-16,0.,-1.));
#113471=DIRECTION('ref_axis',(-1.,0.,1.4081690688991E-16));
#113472=DIRECTION('center_axis',(-1.4081690688991E-16,0.,-1.));
#113473=DIRECTION('ref_axis',(-1.,0.,1.4081690688991E-16));
#113474=DIRECTION('center_axis',(-1.4081690688991E-16,0.,-1.));
#113475=DIRECTION('ref_axis',(-1.,0.,1.4081690688991E-16));
#113476=DIRECTION('',(-0.866025403784445,-0.499999999999989,1.21951018649011E-16));
#113477=DIRECTION('center_axis',(1.4081690688991E-16,0.,1.));
#113478=DIRECTION('ref_axis',(1.,0.,-1.4081690688991E-16));
#113479=DIRECTION('',(0.45677941465413,0.203366068089046,0.866022406579779));
#113480=DIRECTION('center_axis',(1.4081690688991E-16,0.,1.));
#113481=DIRECTION('ref_axis',(-1.,0.,1.40816906889911E-16));
#113482=DIRECTION('',(-0.433014808647733,-0.250006733496379,-0.866022406579782));
#113483=DIRECTION('center_axis',(-1.4081690688991E-16,0.,-1.));
#113484=DIRECTION('ref_axis',(-1.,0.,1.40816906889911E-16));
#113485=DIRECTION('center_axis',(-1.4081690688991E-16,0.,-1.));
#113486=DIRECTION('ref_axis',(-1.,0.,1.4081690688991E-16));
#113487=DIRECTION('',(0.913545457642606,0.406736643075789,-1.2864264564856E-16));
#113488=DIRECTION('center_axis',(1.4081690688991E-16,0.,1.));
#113489=DIRECTION('ref_axis',(-1.,0.,1.4081690688991E-16));
#113490=DIRECTION('',(-0.866025403784445,-0.499999999999989,1.21951018649011E-16));
#113491=DIRECTION('center_axis',(-1.4081690688991E-16,0.,-1.));
#113492=DIRECTION('ref_axis',(-1.,0.,1.4081690688991E-16));
#113493=DIRECTION('center_axis',(-1.4081690688991E-16,0.,-1.));
#113494=DIRECTION('ref_axis',(1.,2.48689957516035E-14,-1.4081690688991E-16));
#113495=DIRECTION('',(0.456775406784114,0.203374579494995,-0.866022521746659));
#113496=DIRECTION('center_axis',(-1.4081690688991E-16,0.,-1.));
#113497=DIRECTION('ref_axis',(-1.,0.,1.4081690688991E-16));
#113498=DIRECTION('center_axis',(-1.4081690688991E-16,0.,-1.));
#113499=DIRECTION('ref_axis',(-1.,0.,1.4081690688991E-16));
#113500=DIRECTION('center_axis',(-1.4081690688991E-16,0.,-1.));
#113501=DIRECTION('ref_axis',(-1.,0.,1.4081690688991E-16));
#113502=DIRECTION('',(-0.433019338752905,-0.249998488182556,0.866022521746654));
#113503=DIRECTION('center_axis',(-1.4081690688991E-16,0.,-1.));
#113504=DIRECTION('ref_axis',(-1.,0.,1.40816906889911E-16));
#113505=DIRECTION('',(0.913545457642606,0.406736643075789,-1.2864264564856E-16));
#113506=DIRECTION('center_axis',(1.4081690688991E-16,0.,1.));
#113507=DIRECTION('ref_axis',(-1.,0.,1.4081690688991E-16));
#113508=DIRECTION('',(-0.866025403784445,-0.499999999999989,1.21951018649011E-16));
#113509=DIRECTION('center_axis',(-1.4081690688991E-16,0.,-1.));
#113510=DIRECTION('ref_axis',(-1.,0.,1.17174841180864E-16));
#113511=DIRECTION('center_axis',(0.407714137590522,-0.913109622086508,7.86457214212551E-6));
#113512=DIRECTION('ref_axis',(4.54394102509795E-6,-6.58403219129936E-6,
-0.999999999968001));
#113513=DIRECTION('center_axis',(-0.499072844768381,0.866560035746482,7.86457218027767E-6));
#113514=DIRECTION('ref_axis',(-0.73488383318754,-0.423232531439995,-0.529924500330454));
#113515=DIRECTION('center_axis',(-1.4081690688991E-16,0.,-1.));
#113516=DIRECTION('ref_axis',(-1.,0.,1.13676889660403E-16));
#113517=DIRECTION('center_axis',(0.407672492122622,-0.913128216118123,-9.77058808687787E-6));
#113518=DIRECTION('ref_axis',(0.798661963255971,0.356563044148554,0.484769908302521));
#113519=DIRECTION('center_axis',(-0.499112366281653,0.866537273133283,-9.77051754275204E-6));
#113520=DIRECTION('ref_axis',(0.757913804263396,0.436552356525734,0.484756336027508));
#113521=DIRECTION('center_axis',(-1.4081690688991E-16,0.,-1.));
#113522=DIRECTION('ref_axis',(-1.,0.,1.15974593313694E-16));
#113523=DIRECTION('center_axis',(-0.404361593575374,0.914599202553397,1.816247957149E-5));
#113524=DIRECTION('ref_axis',(0.791348561788099,0.349880111829978,-0.50134953984396));
#113525=DIRECTION('center_axis',(0.502248501217063,-0.86472333303575,1.81316453019379E-5));
#113526=DIRECTION('ref_axis',(0.749703650686612,0.435432334018008,-0.498340364247967));
#113527=DIRECTION('center_axis',(-1.4081690688991E-16,0.,-1.));
#113528=DIRECTION('ref_axis',(-1.,0.,1.16261524579732E-16));
#113529=DIRECTION('center_axis',(-0.404349235499867,0.914604666185693,1.84940625621926E-5));
#113530=DIRECTION('ref_axis',(0.792949544399534,0.350555095115829,0.498339387691665));
#113531=DIRECTION('center_axis',(0.502260184874653,-0.864716546821256,1.85257140468035E-5));
#113532=DIRECTION('ref_axis',(0.748187385814963,0.434586366990226,0.501348506862849));
#113533=DIRECTION('center_axis',(-1.4081690688991E-16,0.,-1.));
#113534=DIRECTION('ref_axis',(-1.,0.,1.40816906889911E-16));
#113535=DIRECTION('center_axis',(-1.4081690688991E-16,0.,-1.));
#113536=DIRECTION('ref_axis',(-1.,0.,1.4081690688991E-16));
#113537=DIRECTION('',(0.866025403784445,0.499999999999989,-1.21951018649011E-16));
#113538=DIRECTION('center_axis',(-1.4081690688991E-16,0.,-1.));
#113539=DIRECTION('ref_axis',(-1.,0.,1.4081690688991E-16));
#113540=DIRECTION('center_axis',(-1.4081690688991E-16,0.,-1.));
#113541=DIRECTION('ref_axis',(-1.,0.,1.4081690688991E-16));
#113542=DIRECTION('center_axis',(-1.4081690688991E-16,0.,-1.));
#113543=DIRECTION('ref_axis',(-1.,0.,1.4081690688991E-16));
#113544=DIRECTION('',(-0.809016994374955,-0.587785252292463,1.13923270769253E-16));
#113545=DIRECTION('center_axis',(1.4081690688991E-16,0.,1.));
#113546=DIRECTION('ref_axis',(1.,0.,-1.4081690688991E-16));
#113547=DIRECTION('',(0.433019586648924,0.249998457755589,0.866022406579773));
#113548=DIRECTION('center_axis',(1.4081690688991E-16,0.,1.));
#113549=DIRECTION('ref_axis',(-1.,0.,1.40816906889911E-16));
#113550=DIRECTION('',(-0.404509888559955,-0.293899542971717,-0.866022406579777));
#113551=DIRECTION('center_axis',(-1.4081690688991E-16,0.,-1.));
#113552=DIRECTION('ref_axis',(-1.,0.,1.40816906889911E-16));
#113553=DIRECTION('center_axis',(-1.4081690688991E-16,0.,-1.));
#113554=DIRECTION('ref_axis',(-1.,0.,1.4081690688991E-16));
#113555=DIRECTION('',(0.866025403784445,0.499999999999989,-1.21951018649011E-16));
#113556=DIRECTION('center_axis',(1.4081690688991E-16,0.,1.));
#113557=DIRECTION('ref_axis',(-1.,0.,1.4081690688991E-16));
#113558=DIRECTION('',(-0.809016994374955,-0.587785252292463,1.13923270769253E-16));
#113559=DIRECTION('center_axis',(-1.4081690688991E-16,0.,-1.));
#113560=DIRECTION('ref_axis',(-1.,0.,1.4081690688991E-16));
#113561=DIRECTION('center_axis',(-1.4081690688991E-16,0.,-1.));
#113562=DIRECTION('ref_axis',(1.,1.95399252334028E-14,-1.4081690688991E-16));
#113563=DIRECTION('',(0.433014711050255,0.250006503598669,-0.866022521746653));
#113564=DIRECTION('center_axis',(-1.4081690688991E-16,0.,-1.));
#113565=DIRECTION('ref_axis',(-1.,0.,1.4081690688991E-16));
#113566=DIRECTION('center_axis',(-1.4081690688991E-16,0.,-1.));
#113567=DIRECTION('ref_axis',(-1.,0.,1.4081690688991E-16));
#113568=DIRECTION('center_axis',(-1.4081690688991E-16,0.,-1.));
#113569=DIRECTION('ref_axis',(-1.,0.,1.4081690688991E-16));
#113570=DIRECTION('',(-0.404515255718701,-0.293891816351536,0.866022521746651));
#113571=DIRECTION('center_axis',(-1.4081690688991E-16,0.,-1.));
#113572=DIRECTION('ref_axis',(-1.,0.,1.40816906889911E-16));
#113573=DIRECTION('',(0.866025403784445,0.499999999999989,-1.21951018649011E-16));
#113574=DIRECTION('center_axis',(1.4081690688991E-16,0.,1.));
#113575=DIRECTION('ref_axis',(-1.,0.,1.4081690688991E-16));
#113576=DIRECTION('',(-0.809016994374955,-0.587785252292463,1.13923270769253E-16));
#113577=DIRECTION('center_axis',(-1.4081690688991E-16,0.,-1.));
#113578=DIRECTION('ref_axis',(-1.,0.,1.17174841180864E-16));
#113579=DIRECTION('center_axis',(0.500926582476576,-0.865489779781649,7.86457214533227E-6));
#113580=DIRECTION('ref_axis',(5.20726763301671E-6,-6.0729929870304E-6,-0.999999999968002));
#113581=DIRECTION('center_axis',(-0.586919060371622,0.80964561167874,7.8645721780656E-6));
#113582=DIRECTION('ref_axis',(-0.686618216540878,-0.497730297112552,-0.529924500330447));
#113583=DIRECTION('center_axis',(-1.4081690688991E-16,0.,-1.));
#113584=DIRECTION('ref_axis',(-1.,0.,1.13676889660403E-16));
#113585=DIRECTION('center_axis',(0.500887108754481,-0.865512625088804,-9.77059218766514E-6));
#113586=DIRECTION('ref_axis',(0.757015822392063,0.438092662173902,0.484769908304396));
#113587=DIRECTION('center_axis',(-0.586955986038022,0.809618842640579,-9.77052405936867E-6));
#113588=DIRECTION('ref_axis',(0.708129726178679,0.513384442288736,0.48475633602666));
#113589=DIRECTION('center_axis',(-1.4081690688991E-16,0.,-1.));
#113590=DIRECTION('ref_axis',(-1.,0.,1.15974593313694E-16));
#113591=DIRECTION('center_axis',(-0.497748107605369,0.867321636444865,1.81624798484582E-5));
#113592=DIRECTION('ref_axis',(0.750441041150575,0.430681881042595,-0.501349539840671));
#113593=DIRECTION('center_axis',(0.589885332530237,-0.807487024129141,1.81316453652568E-5));
#113594=DIRECTION('ref_axis',(0.700081622914366,0.511412360645375,-0.498340364245875));
#113595=DIRECTION('center_axis',(-1.4081690688991E-16,0.,-1.));
#113596=DIRECTION('ref_axis',(-1.,0.,1.16261524579732E-16));
#113597=DIRECTION('center_axis',(-0.497736388327921,0.867328361920817,1.84940507090592E-5));
#113598=DIRECTION('ref_axis',(0.751962698442014,0.431520514948995,0.498339387696737));
#113599=DIRECTION('center_axis',(0.589896242826456,-0.807479053818753,1.85257236353235E-5));
#113600=DIRECTION('ref_axis',(0.698662091933123,0.51041253507613,0.501348506862033));
#113601=DIRECTION('center_axis',(-1.4081690688991E-16,0.,-1.));
#113602=DIRECTION('ref_axis',(-1.,0.,1.40816906889911E-16));
#113603=DIRECTION('center_axis',(-1.4081690688991E-16,0.,-1.));
#113604=DIRECTION('ref_axis',(-1.,0.,1.4081690688991E-16));
#113605=DIRECTION('',(0.809016994374955,0.587785252292463,-1.13923270769253E-16));
#113606=DIRECTION('center_axis',(-1.4081690688991E-16,0.,-1.));
#113607=DIRECTION('ref_axis',(-1.,0.,1.4081690688991E-16));
#113608=DIRECTION('center_axis',(-1.4081690688991E-16,0.,-1.));
#113609=DIRECTION('ref_axis',(-1.,0.,1.4081690688991E-16));
#113610=DIRECTION('center_axis',(-1.4081690688991E-16,0.,-1.));
#113611=DIRECTION('ref_axis',(-1.,0.,1.4081690688991E-16));
#113612=DIRECTION('',(-0.743144825477402,-0.66913060635885,1.0464735569497E-16));
#113613=DIRECTION('center_axis',(1.4081690688991E-16,0.,1.));
#113614=DIRECTION('ref_axis',(1.,0.,-1.4081690688991E-16));
#113615=DIRECTION('',(0.404515505437166,0.293891812003437,0.86602240657979));
#113616=DIRECTION('center_axis',(1.4081690688991E-16,0.,1.));
#113617=DIRECTION('ref_axis',(-1.,0.,1.40816906889911E-16));
#113618=DIRECTION('',(-0.371573073483918,-0.334572327551858,-0.866022406579788));
#113619=DIRECTION('center_axis',(-1.4081690688991E-16,0.,-1.));
#113620=DIRECTION('ref_axis',(-1.,0.,1.40816906889911E-16));
#113621=DIRECTION('center_axis',(-1.4081690688991E-16,0.,-1.));
#113622=DIRECTION('ref_axis',(-1.,0.,1.4081690688991E-16));
#113623=DIRECTION('',(0.809016994374955,0.587785252292463,-1.13923270769253E-16));
#113624=DIRECTION('center_axis',(1.4081690688991E-16,0.,1.));
#113625=DIRECTION('ref_axis',(-1.,0.,1.4081690688991E-16));
#113626=DIRECTION('',(-0.743144825477402,-0.66913060635885,1.0464735569497E-16));
#113627=DIRECTION('center_axis',(-1.4081690688991E-16,0.,-1.));
#113628=DIRECTION('ref_axis',(-1.,0.,1.4081690688991E-16));
#113629=DIRECTION('center_axis',(-1.4081690688991E-16,0.,-1.));
#113630=DIRECTION('ref_axis',(1.,1.33226762955019E-14,-1.4081690688991E-16));
#113631=DIRECTION('',(0.404509815527881,0.293899304131705,-0.866022521746692));
#113632=DIRECTION('center_axis',(-1.4081690688991E-16,0.,-1.));
#113633=DIRECTION('ref_axis',(-1.,0.,1.4081690688991E-16));
#113634=DIRECTION('center_axis',(-1.4081690688991E-16,0.,-1.));
#113635=DIRECTION('ref_axis',(-1.,0.,1.4081690688991E-16));
#113636=DIRECTION('center_axis',(-1.4081690688991E-16,0.,-1.));
#113637=DIRECTION('ref_axis',(-1.,0.,1.4081690688991E-16));
#113638=DIRECTION('',(-0.371579218892574,-0.334565204279747,0.866022521746655));
#113639=DIRECTION('center_axis',(-1.4081690688991E-16,0.,-1.));
#113640=DIRECTION('ref_axis',(-1.,0.,1.40816906889911E-16));
#113641=DIRECTION('',(0.809016994374955,0.587785252292463,-1.13923270769253E-16));
#113642=DIRECTION('center_axis',(1.4081690688991E-16,0.,1.));
#113643=DIRECTION('ref_axis',(-1.,0.,1.4081690688991E-16));
#113644=DIRECTION('',(-0.743144825477402,-0.66913060635885,1.0464735569497E-16));
#113645=DIRECTION('center_axis',(-1.4081690688991E-16,0.,-1.));
#113646=DIRECTION('ref_axis',(-1.,0.,1.17174841180864E-16));
#113647=DIRECTION('center_axis',(0.588650770899379,-0.80838745033413,7.86457210154094E-6));
#113648=DIRECTION('ref_axis',(5.81354225308953E-6,-5.4954167984505E-6,-0.999999999968002));
#113649=DIRECTION('center_axis',(-0.668334867928659,0.743860540860268,7.86457229484424E-6));
#113650=DIRECTION('ref_axis',(-0.630829867029782,-0.566774825493071,-0.529924500330459));
#113651=DIRECTION('center_axis',(-1.4081690688991E-16,0.,-1.));
#113652=DIRECTION('ref_axis',(-1.,0.,1.13676889660403E-16));
#113653=DIRECTION('center_axis',(0.588613901402245,-0.808414296620591,-9.77058986000007E-6));
#113654=DIRECTION('ref_axis',(0.70707565776309,0.514822445315893,0.484769908304814));
#113655=DIRECTION('center_axis',(-0.668368793188665,0.743830058680116,-9.77051765906954E-6));
#113656=DIRECTION('ref_axis',(0.650587230627793,0.584591780669081,0.484756336026886));
#113657=DIRECTION('center_axis',(-1.4081690688991E-16,0.,-1.));
#113658=DIRECTION('ref_axis',(-1.,0.,1.15974593313694E-16));
#113659=DIRECTION('center_axis',(-0.585681189208067,0.810541512988662,1.81624795712343E-5));
#113660=DIRECTION('ref_axis',(0.701311531422973,0.506765009438398,-0.501349539844273));
#113661=DIRECTION('center_axis',(0.671059256698672,-0.741403718408715,1.81316452494132E-5));
#113662=DIRECTION('ref_axis',(0.642789354376865,0.581789246427105,-0.498340364250735));
#113663=DIRECTION('center_axis',(-1.4081690688991E-16,0.,-1.));
#113664=DIRECTION('ref_axis',(-1.,0.,1.16261524579732E-16));
#113665=DIRECTION('center_axis',(-0.585670237131424,0.810549426621469,1.84940458788945E-5));
#113666=DIRECTION('ref_axis',(0.702737191804646,0.507758105720061,0.498339387696875));
#113667=DIRECTION('center_axis',(0.671069274101679,-0.741394651325084,1.85257263442263E-5));
#113668=DIRECTION('ref_axis',(0.641482109966447,0.580646516615992,0.501348506863948));
#113669=DIRECTION('center_axis',(-1.4081690688991E-16,0.,-1.));
#113670=DIRECTION('ref_axis',(-1.,0.,1.40816906889911E-16));
#113671=DIRECTION('center_axis',(-1.4081690688991E-16,0.,-1.));
#113672=DIRECTION('ref_axis',(-1.,0.,1.4081690688991E-16));
#113673=DIRECTION('',(0.743144825477402,0.66913060635885,-1.0464735569497E-16));
#113674=DIRECTION('center_axis',(-1.4081690688991E-16,0.,-1.));
#113675=DIRECTION('ref_axis',(-1.,0.,1.4081690688991E-16));
#113676=DIRECTION('center_axis',(-1.4081690688991E-16,0.,-1.));
#113677=DIRECTION('ref_axis',(-1.,0.,1.4081690688991E-16));
#113678=DIRECTION('center_axis',(-1.4081690688991E-16,0.,-1.));
#113679=DIRECTION('ref_axis',(-1.,0.,1.4081690688991E-16));
#113680=DIRECTION('',(-0.669130606358867,-0.743144825477386,9.42249022928259E-17));
#113681=DIRECTION('center_axis',(1.4081690688991E-16,0.,1.));
#113682=DIRECTION('ref_axis',(1.,0.,-1.4081690688991E-16));
#113683=DIRECTION('',(0.371579467697561,0.334565226058171,0.866022406579785));
#113684=DIRECTION('center_axis',(1.4081690688991E-16,0.,1.));
#113685=DIRECTION('ref_axis',(-1.,0.,1.40816906889911E-16));
#113686=DIRECTION('',(-0.334565226058175,-0.371579467697537,-0.866022406579794));
#113687=DIRECTION('center_axis',(-1.4081690688991E-16,0.,-1.));
#113688=DIRECTION('ref_axis',(-1.,0.,1.40816906889911E-16));
#113689=DIRECTION('center_axis',(-1.4081690688991E-16,0.,-1.));
#113690=DIRECTION('ref_axis',(-1.,0.,1.4081690688991E-16));
#113691=DIRECTION('',(0.743144825477402,0.66913060635885,-1.0464735569497E-16));
#113692=DIRECTION('center_axis',(1.4081690688991E-16,0.,1.));
#113693=DIRECTION('ref_axis',(-1.,0.,1.4081690688991E-16));
#113694=DIRECTION('',(-0.669130606358867,-0.743144825477386,9.42249022928259E-17));
#113695=DIRECTION('center_axis',(-1.4081690688991E-16,0.,-1.));
#113696=DIRECTION('ref_axis',(-1.,0.,1.4081690688991E-16));
#113697=DIRECTION('center_axis',(-1.4081690688991E-16,0.,-1.));
#113698=DIRECTION('ref_axis',(1.,1.33226762955019E-14,-1.4081690688991E-16));
#113699=DIRECTION('',(0.371573025817597,0.334572082386321,-0.866022521746655));
#113700=DIRECTION('center_axis',(-1.4081690688991E-16,0.,-1.));
#113701=DIRECTION('ref_axis',(-1.,0.,1.4081690688991E-16));
#113702=DIRECTION('center_axis',(-1.4081690688991E-16,0.,-1.));
#113703=DIRECTION('ref_axis',(-1.,0.,1.4081690688991E-16));
#113704=DIRECTION('center_axis',(-1.4081690688991E-16,0.,-1.));
#113705=DIRECTION('ref_axis',(-1.,0.,1.4081690688991E-16));
#113706=DIRECTION('',(-0.334572082386318,-0.371573025817621,0.866022521746647));
#113707=DIRECTION('center_axis',(-1.4081690688991E-16,0.,-1.));
#113708=DIRECTION('ref_axis',(-1.,0.,1.40816906889911E-16));
#113709=DIRECTION('',(0.743144825477402,0.66913060635885,-1.0464735569497E-16));
#113710=DIRECTION('center_axis',(1.4081690688991E-16,0.,1.));
#113711=DIRECTION('ref_axis',(-1.,0.,1.4081690688991E-16));
#113712=DIRECTION('',(-0.669130606358867,-0.743144825477386,9.42249022928259E-17));
#113713=DIRECTION('center_axis',(-1.4081690688991E-16,0.,-1.));
#113714=DIRECTION('ref_axis',(-1.,0.,1.17174841180864E-16));
#113715=DIRECTION('center_axis',(0.669925578293215,-0.742428258814715,7.86457222451189E-6));
#113716=DIRECTION('ref_axis',(6.35612261558566E-6,-4.85763178434958E-6,
-0.999999999968002));
#113717=DIRECTION('center_axis',(-0.742428258814657,0.66992557829328,7.86457232160625E-6));
#113718=DIRECTION('ref_axis',(-0.568130013485826,-0.629609650280326,-0.529924500330453));
#113719=DIRECTION('center_axis',(-1.4081690688991E-16,0.,-1.));
#113720=DIRECTION('ref_axis',(-1.,0.,1.13676889660403E-16));
#113721=DIRECTION('center_axis',(0.669891716970495,-0.742458811947746,-9.77058614774733E-6));
#113722=DIRECTION('ref_axis',(0.649388624263242,0.585911726014071,0.484769908303626));
#113723=DIRECTION('center_axis',(-0.742458811969737,0.669891716946122,-9.77052681755937E-6));
#113724=DIRECTION('ref_axis',(0.585916765233622,0.649394209166309,0.484756336028146));
#113725=DIRECTION('center_axis',(-1.4081690688991E-16,0.,-1.));
#113726=DIRECTION('ref_axis',(-1.,0.,1.15974593313694E-16));
#113727=DIRECTION('center_axis',(-0.667197425140104,0.744880927099453,1.81624795753533E-5));
#113728=DIRECTION('ref_axis',(0.644498305802597,0.577295914346879,-0.501349539838209));
#113729=DIRECTION('center_axis',(0.744880915222603,-0.667197438400643,1.8131645392797E-5));
#113730=DIRECTION('ref_axis',(0.578454551163898,0.645791927480607,-0.498340364247827));
#113731=DIRECTION('center_axis',(-1.4081690688991E-16,0.,-1.));
#113732=DIRECTION('ref_axis',(-1.,0.,1.16261524579732E-16));
#113733=DIRECTION('center_axis',(-0.667187360268565,0.744889942176584,1.8494066007285E-5));
#113734=DIRECTION('ref_axis',(0.645812349439158,0.578432592431863,0.498339387691189));
#113735=DIRECTION('center_axis',(0.744889929979156,-0.667187373885662,1.85257309138967E-5));
#113736=DIRECTION('ref_axis',(0.577273915764732,0.644518813412092,0.501348506864758));
#113737=DIRECTION('center_axis',(-1.4081690688991E-16,0.,-1.));
#113738=DIRECTION('ref_axis',(-1.,0.,1.40816906889911E-16));
#113739=DIRECTION('center_axis',(-1.4081690688991E-16,0.,-1.));
#113740=DIRECTION('ref_axis',(-1.,0.,1.4081690688991E-16));
#113741=DIRECTION('',(0.669130606358867,0.743144825477386,-9.42249022928259E-17));
#113742=DIRECTION('center_axis',(-1.4081690688991E-16,0.,-1.));
#113743=DIRECTION('ref_axis',(-1.,0.,1.4081690688991E-16));
#113744=DIRECTION('center_axis',(-1.4081690688991E-16,0.,-1.));
#113745=DIRECTION('ref_axis',(-1.,0.,1.4081690688991E-16));
#113746=DIRECTION('center_axis',(-1.4081690688991E-16,0.,-1.));
#113747=DIRECTION('ref_axis',(-1.,0.,1.4081690688991E-16));
#113748=DIRECTION('',(-0.587785252292482,-0.809016994374941,8.2770101143333E-17));
#113749=DIRECTION('center_axis',(1.4081690688991E-16,0.,1.));
#113750=DIRECTION('ref_axis',(1.,0.,-1.4081690688991E-16));
#113751=DIRECTION('',(0.334572327551885,0.371573073483891,0.866022406579789));
#113752=DIRECTION('center_axis',(1.4081690688991E-16,0.,1.));
#113753=DIRECTION('ref_axis',(-1.,1.86517468137026E-14,1.40816906889911E-16));
#113754=DIRECTION('',(-0.293891812003428,-0.404515505437145,-0.866022406579803));
#113755=DIRECTION('center_axis',(-1.4081690688991E-16,0.,-1.));
#113756=DIRECTION('ref_axis',(-1.,0.,1.40816906889911E-16));
#113757=DIRECTION('center_axis',(-1.4081690688991E-16,0.,-1.));
#113758=DIRECTION('ref_axis',(-1.,0.,1.4081690688991E-16));
#113759=DIRECTION('',(0.669130606358867,0.743144825477386,-9.42249022928259E-17));
#113760=DIRECTION('center_axis',(1.4081690688991E-16,0.,1.));
#113761=DIRECTION('ref_axis',(-1.,1.86517468137026E-14,1.4081690688991E-16));
#113762=DIRECTION('',(-0.587785252292482,-0.809016994374941,8.2770101143333E-17));
#113763=DIRECTION('center_axis',(-1.4081690688991E-16,0.,-1.));
#113764=DIRECTION('ref_axis',(-1.,0.,1.4081690688991E-16));
#113765=DIRECTION('center_axis',(-1.4081690688991E-16,0.,-1.));
#113766=DIRECTION('ref_axis',(1.,-2.66453525910038E-14,-1.4081690688991E-16));
#113767=DIRECTION('',(0.33456520427975,0.371579218892551,-0.866022521746664));
#113768=DIRECTION('center_axis',(-1.4081690688991E-16,0.,-1.));
#113769=DIRECTION('ref_axis',(-1.,0.,1.4081690688991E-16));
#113770=DIRECTION('center_axis',(-1.4081690688991E-16,0.,-1.));
#113771=DIRECTION('ref_axis',(-1.,0.,1.4081690688991E-16));
#113772=DIRECTION('center_axis',(-1.4081690688991E-16,0.,-1.));
#113773=DIRECTION('ref_axis',(-1.,0.,1.4081690688991E-16));
#113774=DIRECTION('',(-0.293899304131723,-0.404509815527924,0.866022521746666));
#113775=DIRECTION('center_axis',(-1.4081690688991E-16,0.,-1.));
#113776=DIRECTION('ref_axis',(-1.,0.,1.40816906889911E-16));
#113777=DIRECTION('',(0.669130606358867,0.743144825477386,-9.42249022928259E-17));
#113778=DIRECTION('center_axis',(1.4081690688991E-16,0.,1.));
#113779=DIRECTION('ref_axis',(-1.,0.,1.4081690688991E-16));
#113780=DIRECTION('',(-0.587785252292482,-0.809016994374941,8.2770101143333E-17));
#113781=DIRECTION('center_axis',(-1.4081690688991E-16,0.,-1.));
#113782=DIRECTION('ref_axis',(-1.,0.,1.17174841180864E-16));
#113783=DIRECTION('center_axis',(0.743860540860151,-0.66833486792879,7.86457201063913E-6));
#113784=DIRECTION('ref_axis',(6.82906374699039E-6,-4.16662528541481E-6,
-0.999999999968002));
#113785=DIRECTION('center_axis',(-0.808387450334093,0.58865077089943,7.86457218447997E-6));
#113786=DIRECTION('ref_axis',(-0.499205608625081,-0.685546339984944,-0.529924500330481));
#113787=DIRECTION('center_axis',(-1.4081690688991E-16,0.,-1.));
#113788=DIRECTION('ref_axis',(-1.,0.,1.13676889660403E-16));
#113789=DIRECTION('center_axis',(0.743830058703253,-0.668368793162915,-9.77058023976066E-6));
#113790=DIRECTION('ref_axis',(0.584586753102912,0.650581635232641,0.484769908301471));
#113791=DIRECTION('center_axis',(-0.808414296642385,0.588613901372314,-9.77052295710416E-6));
#113792=DIRECTION('ref_axis',(0.5148268731491,0.707081738813847,0.484756336028222));
#113793=DIRECTION('center_axis',(-1.4081690688991E-16,0.,-1.));
#113794=DIRECTION('ref_axis',(-1.,0.,1.15974593313694E-16));
#113795=DIRECTION('center_axis',(-0.741403706462291,0.671059269896558,1.8162479572778E-5));
#113796=DIRECTION('ref_axis',(0.58062382187003,0.641501844407687,-0.501349539840793));
#113797=DIRECTION('center_axis',(0.810541502562919,-0.585681203637515,1.81316451184131E-5));
#113798=DIRECTION('ref_axis',(0.507782078838013,0.702719177035393,-0.498340364246813));
#113799=DIRECTION('center_axis',(-1.4081690688991E-16,0.,-1.));
#113800=DIRECTION('ref_axis',(-1.,0.,1.16261524579732E-16));
#113801=DIRECTION('center_axis',(-0.741394639060127,0.671069287652828,1.84940680536415E-5));
#113802=DIRECTION('ref_axis',(0.581811851823624,0.642769650612115,0.498339387696322));
#113803=DIRECTION('center_axis',(0.810549415916517,-0.585670251945744,1.85257039599468E-5));
#113804=DIRECTION('ref_axis',(0.506740987741176,0.701329627215963,0.501348506861461));
#113805=DIRECTION('center_axis',(-1.4081690688991E-16,0.,-1.));
#113806=DIRECTION('ref_axis',(-1.,0.,1.40816906889911E-16));
#113807=DIRECTION('center_axis',(-1.4081690688991E-16,0.,-1.));
#113808=DIRECTION('ref_axis',(-1.,0.,1.4081690688991E-16));
#113809=DIRECTION('',(0.587785252292482,0.809016994374941,-8.2770101143333E-17));
#113810=DIRECTION('center_axis',(-1.4081690688991E-16,0.,-1.));
#113811=DIRECTION('ref_axis',(-1.,0.,1.4081690688991E-16));
#113812=DIRECTION('center_axis',(-1.4081690688991E-16,0.,-1.));
#113813=DIRECTION('ref_axis',(-1.,0.,1.4081690688991E-16));
#113814=DIRECTION('center_axis',(-1.4081690688991E-16,0.,-1.));
#113815=DIRECTION('ref_axis',(-1.,0.,1.4081690688991E-16));
#113816=DIRECTION('',(-0.50000000000001,-0.866025403784433,7.04084534449566E-17));
#113817=DIRECTION('center_axis',(1.4081690688991E-16,0.,1.));
#113818=DIRECTION('ref_axis',(1.,0.,-1.4081690688991E-16));
#113819=DIRECTION('',(0.293899542971749,0.404509888559906,0.866022406579789));
#113820=DIRECTION('center_axis',(1.4081690688991E-16,0.,1.));
#113821=DIRECTION('ref_axis',(-1.,-1.95399252334028E-14,1.40816906889911E-16));
#113822=DIRECTION('',(-0.249998457755608,-0.433019586648879,-0.866022406579791));
#113823=DIRECTION('center_axis',(-1.4081690688991E-16,0.,-1.));
#113824=DIRECTION('ref_axis',(-1.,0.,1.40816906889911E-16));
#113825=DIRECTION('center_axis',(-1.4081690688991E-16,0.,-1.));
#113826=DIRECTION('ref_axis',(-1.,0.,1.4081690688991E-16));
#113827=DIRECTION('',(0.587785252292482,0.809016994374941,-8.2770101143333E-17));
#113828=DIRECTION('center_axis',(1.4081690688991E-16,0.,1.));
#113829=DIRECTION('ref_axis',(-1.,-1.86517468137026E-14,1.4081690688991E-16));
#113830=DIRECTION('',(-0.50000000000001,-0.866025403784433,7.04084534449566E-17));
#113831=DIRECTION('center_axis',(-1.4081690688991E-16,0.,-1.));
#113832=DIRECTION('ref_axis',(-1.,0.,1.4081690688991E-16));
#113833=DIRECTION('center_axis',(-1.4081690688991E-16,0.,-1.));
#113834=DIRECTION('ref_axis',(1.,1.24344978758018E-14,-1.4081690688991E-16));
#113835=DIRECTION('',(0.293891816351536,0.404515255718701,-0.866022521746651));
#113836=DIRECTION('center_axis',(-1.4081690688991E-16,0.,-1.));
#113837=DIRECTION('ref_axis',(-1.,0.,1.4081690688991E-16));
#113838=DIRECTION('center_axis',(-1.4081690688991E-16,0.,-1.));
#113839=DIRECTION('ref_axis',(-1.,0.,1.4081690688991E-16));
#113840=DIRECTION('center_axis',(-1.4081690688991E-16,0.,-1.));
#113841=DIRECTION('ref_axis',(-1.,0.,1.4081690688991E-16));
#113842=DIRECTION('',(-0.250006503598682,-0.433014711050253,0.86602252174665));
#113843=DIRECTION('center_axis',(-1.4081690688991E-16,0.,-1.));
#113844=DIRECTION('ref_axis',(-1.,0.,1.40816906889911E-16));
#113845=DIRECTION('',(0.587785252292482,0.809016994374941,-8.2770101143333E-17));
#113846=DIRECTION('center_axis',(1.4081690688991E-16,0.,1.));
#113847=DIRECTION('ref_axis',(-1.,1.95399252334028E-14,1.4081690688991E-16));
#113848=DIRECTION('',(-0.50000000000001,-0.866025403784433,7.04084534449566E-17));
#113849=DIRECTION('center_axis',(-1.4081690688991E-16,0.,-1.));
#113850=DIRECTION('ref_axis',(-1.,0.,1.17174841180864E-16));
#113851=DIRECTION('center_axis',(0.809645611678693,-0.586919060371687,7.86457198631099E-6));
#113852=DIRECTION('ref_axis',(7.2271843168904E-6,-3.42996854670039E-6,-0.999999999968002));
#113853=DIRECTION('center_axis',(-0.865489779781559,0.50092658247673,7.86457232116346E-6));
#113854=DIRECTION('ref_axis',(-0.424811802651054,-0.733972040528688,-0.529924500330486));
#113855=DIRECTION('center_axis',(-1.4081690688991E-16,0.,-1.));
#113856=DIRECTION('ref_axis',(-1.,0.,1.13676889660403E-16));
#113857=DIRECTION('center_axis',(0.80961884265869,-0.58695598601304,-9.77057981626784E-6));
#113858=DIRECTION('ref_axis',(0.513380027140866,0.70812363591017,0.484769908305172));
#113859=DIRECTION('center_axis',(-0.865512625109973,0.500887108717902,-9.77051588858328E-6));
#113860=DIRECTION('ref_axis',(0.438096430107544,0.757022332963905,0.484756336029672));
#113861=DIRECTION('center_axis',(-1.4081690688991E-16,0.,-1.));
#113862=DIRECTION('ref_axis',(-1.,0.,1.15974593313694E-16));
#113863=DIRECTION('center_axis',(-0.807487013627686,0.589885346904605,1.81624797272146E-5));
#113864=DIRECTION('ref_axis',(0.510387901841611,0.698679346017535,-0.501349539844436));
#113865=DIRECTION('center_axis',(0.867321627584511,-0.497748123045581,1.81316451958916E-5));
#113866=DIRECTION('ref_axis',(0.431546239794257,0.751947288229924,-0.498340364252286));
#113867=DIRECTION('center_axis',(-1.4081690688991E-16,0.,-1.));
#113868=DIRECTION('ref_axis',(-1.,0.,1.16261524579732E-16));
#113869=DIRECTION('center_axis',(-0.80747904303877,0.589896257583621,1.84940691754006E-5));
#113870=DIRECTION('ref_axis',(0.511436901809337,0.7000643899933,0.498339387697757));
#113871=DIRECTION('center_axis',(0.867328352817319,-0.497736404190002,1.85257287627715E-5));
#113872=DIRECTION('ref_axis',(0.43065609941129,0.750456526858726,0.501348506864229));
#113873=DIRECTION('center_axis',(-1.4081690688991E-16,0.,-1.));
#113874=DIRECTION('ref_axis',(-1.,0.,1.40816906889911E-16));
#113875=DIRECTION('center_axis',(-1.4081690688991E-16,0.,-1.));
#113876=DIRECTION('ref_axis',(-1.,0.,1.4081690688991E-16));
#113877=DIRECTION('',(0.50000000000001,0.866025403784433,-7.04084534449566E-17));
#113878=DIRECTION('center_axis',(-1.4081690688991E-16,0.,-1.));
#113879=DIRECTION('ref_axis',(-1.,0.,1.4081690688991E-16));
#113880=DIRECTION('center_axis',(-1.4081690688991E-16,0.,-1.));
#113881=DIRECTION('ref_axis',(-1.,0.,1.4081690688991E-16));
#113882=DIRECTION('center_axis',(-1.4081690688991E-16,0.,-1.));
#113883=DIRECTION('ref_axis',(-1.,0.,1.4081690688991E-16));
#113884=DIRECTION('',(-0.40673664307581,-0.913545457642596,5.72753959967212E-17));
#113885=DIRECTION('center_axis',(1.4081690688991E-16,0.,1.));
#113886=DIRECTION('ref_axis',(1.,0.,-1.4081690688991E-16));
#113887=DIRECTION('',(0.250006733496405,0.43301480864773,0.866022406579776));
#113888=DIRECTION('center_axis',(1.4081690688991E-16,0.,1.));
#113889=DIRECTION('ref_axis',(-1.,-3.90798504668055E-14,1.40816906889911E-16));
#113890=DIRECTION('',(-0.203366068089036,-0.456779414654109,-0.866022406579792));
#113891=DIRECTION('center_axis',(-1.4081690688991E-16,0.,-1.));
#113892=DIRECTION('ref_axis',(-1.,0.,1.40816906889911E-16));
#113893=DIRECTION('center_axis',(-1.4081690688991E-16,0.,-1.));
#113894=DIRECTION('ref_axis',(-1.,0.,1.4081690688991E-16));
#113895=DIRECTION('',(0.50000000000001,0.866025403784433,-7.04084534449566E-17));
#113896=DIRECTION('center_axis',(1.4081690688991E-16,0.,1.));
#113897=DIRECTION('ref_axis',(-1.,-4.08562073062058E-14,1.4081690688991E-16));
#113898=DIRECTION('',(-0.40673664307581,-0.913545457642596,5.72753959967212E-17));
#113899=DIRECTION('center_axis',(-1.4081690688991E-16,0.,-1.));
#113900=DIRECTION('ref_axis',(-1.,0.,1.4081690688991E-16));
#113901=DIRECTION('center_axis',(-1.4081690688991E-16,0.,-1.));
#113902=DIRECTION('ref_axis',(1.,1.24344978758018E-14,-1.4081690688991E-16));
#113903=DIRECTION('',(0.249998488182559,0.433019338752883,-0.866022521746664));
#113904=DIRECTION('center_axis',(-1.4081690688991E-16,0.,-1.));
#113905=DIRECTION('ref_axis',(-1.,0.,1.4081690688991E-16));
#113906=DIRECTION('center_axis',(-1.4081690688991E-16,0.,-1.));
#113907=DIRECTION('ref_axis',(-1.,0.,1.4081690688991E-16));
#113908=DIRECTION('center_axis',(-1.4081690688991E-16,0.,-1.));
#113909=DIRECTION('ref_axis',(-1.,0.,1.4081690688991E-16));
#113910=DIRECTION('',(-0.203374579494995,-0.456775406784114,0.866022521746659));
#113911=DIRECTION('center_axis',(-1.4081690688991E-16,0.,-1.));
#113912=DIRECTION('ref_axis',(-1.,0.,1.40816906889911E-16));
#113913=DIRECTION('',(0.50000000000001,0.866025403784433,-7.04084534449566E-17));
#113914=DIRECTION('center_axis',(1.4081690688991E-16,0.,1.));
#113915=DIRECTION('ref_axis',(-1.,3.90798504668055E-14,1.4081690688991E-16));
#113916=DIRECTION('',(-0.40673664307581,-0.913545457642596,5.72753959967212E-17));
#113917=DIRECTION('center_axis',(-1.4081690688991E-16,0.,-1.));
#113918=DIRECTION('ref_axis',(-1.,0.,1.17174841180864E-16));
#113919=DIRECTION('center_axis',(0.866560035746456,-0.499072844768427,7.86457212100347E-6));
#113920=DIRECTION('ref_axis',(7.54612252965279E-6,-2.65573237658704E-6,
-0.999999999968001));
#113921=DIRECTION('center_axis',(-0.913109622086468,0.407714137590612,7.86457225083087E-6));
#113922=DIRECTION('ref_axis',(-0.345763669669355,-0.774356189803036,-0.529924500330477));
#113923=DIRECTION('center_axis',(-1.4081690688991E-16,0.,-1.));
#113924=DIRECTION('ref_axis',(-1.,0.,1.13676889660403E-16));
#113925=DIRECTION('center_axis',(0.866537273151611,-0.499112366249832,-9.77058386824003E-6));
#113926=DIRECTION('ref_axis',(0.436548602171663,0.757907285850706,0.484769908303293));
#113927=DIRECTION('center_axis',(-0.913128216134471,0.407672492086008,-9.77051561494199E-6));
#113928=DIRECTION('ref_axis',(0.356566110901319,0.798668832019173,0.484756336026502));
#113929=DIRECTION('center_axis',(-1.4081690688991E-16,0.,-1.));
#113930=DIRECTION('ref_axis',(-1.,0.,1.15974593313694E-16));
#113931=DIRECTION('center_axis',(-0.864723324094313,0.502248516610458,1.81624798191131E-5));
#113932=DIRECTION('ref_axis',(0.434560065158887,0.748201970510128,-0.501349539836096));
#113933=DIRECTION('center_axis',(0.914599195355562,-0.404361609857071,1.81316452823751E-5));
#113934=DIRECTION('ref_axis',(0.350582289841991,0.792936907581347,-0.498340364253665));
#113935=DIRECTION('center_axis',(-1.4081690688991E-16,0.,-1.));
#113936=DIRECTION('ref_axis',(-1.,0.,1.16261524579732E-16));
#113937=DIRECTION('center_axis',(-0.864716537640355,0.502260200682123,1.84940508031252E-5));
#113938=DIRECTION('ref_axis',(0.435458542075013,0.7496890774218,0.498339387695128));
#113939=DIRECTION('center_axis',(0.914604658800418,-0.404349252203302,1.85256963593625E-5));
#113940=DIRECTION('ref_axis',(0.34985285273782,0.791361267753626,0.501348506859832));
#113941=DIRECTION('center_axis',(-1.4081690688991E-16,0.,-1.));
#113942=DIRECTION('ref_axis',(-1.,0.,1.40816906889911E-16));
#113943=DIRECTION('center_axis',(-1.4081690688991E-16,0.,-1.));
#113944=DIRECTION('ref_axis',(-1.,0.,1.4081690688991E-16));
#113945=DIRECTION('',(0.40673664307581,0.913545457642596,-5.72753959967212E-17));
#113946=DIRECTION('center_axis',(-1.4081690688991E-16,0.,-1.));
#113947=DIRECTION('ref_axis',(-1.,0.,1.4081690688991E-16));
#113948=DIRECTION('center_axis',(-1.4081690688991E-16,0.,-1.));
#113949=DIRECTION('ref_axis',(-1.,0.,1.4081690688991E-16));
#113950=DIRECTION('center_axis',(-1.4081690688991E-16,0.,-1.));
#113951=DIRECTION('ref_axis',(-1.,0.,1.4081690688991E-16));
#113952=DIRECTION('',(-0.309016994374957,-0.95105651629515,4.35148173242984E-17));
#113953=DIRECTION('center_axis',(1.4081690688991E-16,0.,1.));
#113954=DIRECTION('ref_axis',(1.,0.,-1.4081690688991E-16));
#113955=DIRECTION('',(0.203374797931567,0.456775527877826,0.866022406579776));
#113956=DIRECTION('center_axis',(1.4081690688991E-16,0.,1.));
#113957=DIRECTION('ref_axis',(-1.,-9.76996261670138E-15,1.40816906889911E-16));
#113958=DIRECTION('',(-0.154505557223409,-0.475534671805168,-0.866022406579781));
#113959=DIRECTION('center_axis',(-1.4081690688991E-16,0.,-1.));
#113960=DIRECTION('ref_axis',(-1.,0.,1.40816906889911E-16));
#113961=DIRECTION('center_axis',(-1.4081690688991E-16,0.,-1.));
#113962=DIRECTION('ref_axis',(-1.,0.,1.4081690688991E-16));
#113963=DIRECTION('',(0.40673664307581,0.913545457642596,-5.72753959967212E-17));
#113964=DIRECTION('center_axis',(1.4081690688991E-16,0.,1.));
#113965=DIRECTION('ref_axis',(-1.,-9.76996261670138E-15,1.4081690688991E-16));
#113966=DIRECTION('',(-0.309016994374957,-0.95105651629515,4.35148173242984E-17));
#113967=DIRECTION('center_axis',(-1.4081690688991E-16,0.,-1.));
#113968=DIRECTION('ref_axis',(-1.,0.,1.4081690688991E-16));
#113969=DIRECTION('center_axis',(-1.4081690688991E-16,0.,-1.));
#113970=DIRECTION('ref_axis',(1.,1.24344978758018E-14,-1.4081690688991E-16));
#113971=DIRECTION('',(0.203366124261493,0.45677917129659,-0.866022521746669));
#113972=DIRECTION('center_axis',(-1.4081690688991E-16,0.,-1.));
#113973=DIRECTION('ref_axis',(-1.,0.,1.4081690688991E-16));
#113974=DIRECTION('center_axis',(-1.4081690688991E-16,0.,-1.));
#113975=DIRECTION('ref_axis',(-1.,0.,1.4081690688991E-16));
#113976=DIRECTION('center_axis',(-1.4081690688991E-16,0.,-1.));
#113977=DIRECTION('ref_axis',(-1.,0.,1.4081690688991E-16));
#113978=DIRECTION('',(-0.154514440939481,-0.475531575574859,0.866022521746664));
#113979=DIRECTION('center_axis',(-1.4081690688991E-16,0.,-1.));
#113980=DIRECTION('ref_axis',(-1.,0.,1.40816906889911E-16));
#113981=DIRECTION('',(0.40673664307581,0.913545457642596,-5.72753959967212E-17));
#113982=DIRECTION('center_axis',(1.4081690688991E-16,0.,1.));
#113983=DIRECTION('ref_axis',(-1.,0.,1.4081690688991E-16));
#113984=DIRECTION('',(-0.309016994374957,-0.95105651629515,4.35148173242984E-17));
#113985=DIRECTION('center_axis',(-1.4081690688991E-16,0.,-1.));
#113986=DIRECTION('ref_axis',(-1.,0.,1.17174841180864E-16));
#113987=DIRECTION('center_axis',(0.913980246723209,-0.405758682640226,7.86457201705324E-6));
#113988=DIRECTION('ref_axis',(7.78238360297463E-6,-1.85239937195232E-6,
-0.999999999968002));
#113989=DIRECTION('center_axis',(-0.950725244291279,0.310034691293469,7.86457228312283E-6));
#113990=DIRECTION('ref_axis',(-0.262927277567183,-0.806256330617375,-0.529924500330486));
#113991=DIRECTION('center_axis',(-1.4081690688991E-16,0.,-1.));
#113992=DIRECTION('ref_axis',(-1.,0.,1.13676889660403E-16));
#113993=DIRECTION('center_axis',(0.913961739943276,-0.405800366959415,-9.7705808297001E-6));
#113994=DIRECTION('ref_axis',(0.354934259363254,0.799387144965269,0.484769908301385));
#113995=DIRECTION('center_axis',(-0.950739383338138,0.309991330321275,-9.77051799119866E-6));
#113996=DIRECTION('ref_axis',(0.271129178766797,0.831564948216653,0.484756336027367));
#113997=DIRECTION('center_axis',(-1.4081690688991E-16,0.,-1.));
#113998=DIRECTION('ref_axis',(-1.,0.,1.15974593313694E-16));
#113999=DIRECTION('center_axis',(-0.912485544867192,0.409108946466033,1.81624796700739E-5));
#114000=DIRECTION('ref_axis',(0.353971097458838,0.789527137631561,-0.501349539849295));
#114001=DIRECTION('center_axis',(0.951856222950106,-0.30654482625287,1.81316452438961E-5));
#114002=DIRECTION('ref_axis',(0.265777286960435,0.825238944247301,-0.498340364242704));
#114003=DIRECTION('center_axis',(-1.4081690688991E-16,0.,-1.));
#114004=DIRECTION('ref_axis',(-1.,0.,1.16261524579732E-16));
#114005=DIRECTION('center_axis',(-0.91248001690956,0.409121275905689,1.84940567058976E-5));
#114006=DIRECTION('ref_axis',(0.354709207426606,0.791100014432689,0.498339387698172));
#114007=DIRECTION('center_axis',(0.951860364736293,-0.306531965218784,1.85257121801136E-5));
#114008=DIRECTION('ref_axis',(0.265216544996555,0.823595688992732,0.501348506861921));
#114009=DIRECTION('center_axis',(-1.4081690688991E-16,0.,-1.));
#114010=DIRECTION('ref_axis',(-1.,0.,1.40816906889911E-16));
#114011=DIRECTION('center_axis',(-1.4081690688991E-16,0.,-1.));
#114012=DIRECTION('ref_axis',(-1.,0.,1.4081690688991E-16));
#114013=DIRECTION('',(0.309016994374957,0.95105651629515,-4.35148173242984E-17));
#114014=DIRECTION('center_axis',(-1.4081690688991E-16,0.,-1.));
#114015=DIRECTION('ref_axis',(-1.,0.,1.4081690688991E-16));
#114016=DIRECTION('center_axis',(-1.4081690688991E-16,0.,-1.));
#114017=DIRECTION('ref_axis',(-1.,0.,1.4081690688991E-16));
#114018=DIRECTION('center_axis',(-1.4081690688991E-16,0.,-1.));
#114019=DIRECTION('ref_axis',(-1.,0.,1.4081690688991E-16));
#114020=DIRECTION('',(-0.20791169081777,-0.978147600733803,2.92774812072098E-17));
#114021=DIRECTION('center_axis',(1.4081690688991E-16,0.,1.));
#114022=DIRECTION('ref_axis',(1.,0.,-1.4081690688991E-16));
#114023=DIRECTION('',(0.154514645521724,0.475531718838029,0.866022406579787));
#114024=DIRECTION('center_axis',(1.4081690688991E-16,0.,1.));
#114025=DIRECTION('ref_axis',(-1.,3.10862446895044E-14,1.40816906889911E-16));
#114026=DIRECTION('',(-0.103952251140494,-0.489079871579877,-0.86602240657978));
#114027=DIRECTION('center_axis',(-1.4081690688991E-16,0.,-1.));
#114028=DIRECTION('ref_axis',(-1.,0.,1.40816906889911E-16));
#114029=DIRECTION('center_axis',(-1.4081690688991E-16,0.,-1.));
#114030=DIRECTION('ref_axis',(-1.,0.,1.4081690688991E-16));
#114031=DIRECTION('',(0.309016994374957,0.95105651629515,-4.35148173242984E-17));
#114032=DIRECTION('center_axis',(1.4081690688991E-16,0.,1.));
#114033=DIRECTION('ref_axis',(-1.,3.10862446895044E-14,1.4081690688991E-16));
#114034=DIRECTION('',(-0.20791169081777,-0.978147600733803,2.92774812072098E-17));
#114035=DIRECTION('center_axis',(-1.4081690688991E-16,0.,-1.));
#114036=DIRECTION('ref_axis',(-1.,0.,1.4081690688991E-16));
#114037=DIRECTION('center_axis',(-1.4081690688991E-16,0.,-1.));
#114038=DIRECTION('ref_axis',(1.,-3.5527136788005E-14,-1.4081690688991E-16));
#114039=DIRECTION('',(0.154505638525956,0.475534435652422,-0.866022521746646));
#114040=DIRECTION('center_axis',(-1.4081690688991E-16,0.,-1.));
#114041=DIRECTION('ref_axis',(-1.,0.,1.4081690688991E-16));
#114042=DIRECTION('center_axis',(-1.4081690688991E-16,0.,-1.));
#114043=DIRECTION('ref_axis',(-1.,0.,1.4081690688991E-16));
#114044=DIRECTION('center_axis',(-1.4081690688991E-16,0.,-1.));
#114045=DIRECTION('ref_axis',(-1.,0.,1.4081690688991E-16));
#114046=DIRECTION('',(-0.103961409834817,-0.489077720912241,0.866022521746661));
#114047=DIRECTION('center_axis',(-1.4081690688991E-16,0.,-1.));
#114048=DIRECTION('ref_axis',(-1.,0.,1.40816906889911E-16));
#114049=DIRECTION('',(0.309016994374957,0.95105651629515,-4.35148173242984E-17));
#114050=DIRECTION('center_axis',(1.4081690688991E-16,0.,1.));
#114051=DIRECTION('ref_axis',(-1.,0.,1.4081690688991E-16));
#114052=DIRECTION('',(-0.20791169081777,-0.978147600733803,2.92774812072098E-17));
#114053=DIRECTION('center_axis',(-1.4081690688991E-16,0.,-1.));
#114054=DIRECTION('ref_axis',(-1.,0.,1.17174841180864E-16));
#114055=DIRECTION('center_axis',(0.951386698854214,-0.307998943474534,7.86457199139798E-6));
#114056=DIRECTION('ref_axis',(7.93337931586199E-6,-1.02877117099849E-6,
-0.999999999968002));
#114057=DIRECTION('center_axis',(-0.977924521767597,0.208958440039556,7.86457226078363E-6));
#114058=DIRECTION('ref_axis',(-0.177210199190864,-0.829322958353517,-0.529924500330476));
#114059=DIRECTION('center_axis',(-1.4081690688991E-16,0.,-1.));
#114060=DIRECTION('ref_axis',(-1.,0.,1.13676889660403E-16));
#114061=DIRECTION('center_axis',(0.951372650655522,-0.308042333923799,-9.77058865439169E-6));
#114062=DIRECTION('ref_axis',(0.269431182533645,0.832108751235234,0.484769908303168));
#114063=DIRECTION('center_axis',(-0.977934050903654,0.208913838669691,-9.77051656141964E-6));
#114064=DIRECTION('ref_axis',(0.182721698612562,0.855350264826251,0.484756336026464));
#114065=DIRECTION('center_axis',(-1.4081690688991E-16,0.,-1.));
#114066=DIRECTION('ref_axis',(-1.,0.,1.15974593313694E-16));
#114067=DIRECTION('center_axis',(-0.950250383060598,0.311487093092654,1.81624798101011E-5));
#114068=DIRECTION('ref_axis',(0.269503948347349,0.822202080225929,-0.501349539839565));
#114069=DIRECTION('center_axis',(0.978684514577293,-0.205369473383585,1.8131645285516E-5));
#114070=DIRECTION('ref_axis',(0.178060372502838,0.848499490341508,-0.498340364243508));
#114071=DIRECTION('center_axis',(-1.4081690688991E-16,0.,-1.));
#114072=DIRECTION('ref_axis',(-1.,0.,1.16261524579732E-16));
#114073=DIRECTION('center_axis',(-0.950246174164386,0.311499932815269,1.84940638835828E-5));
#114074=DIRECTION('ref_axis',(0.270073604474708,0.82384349413839,0.498339387698673));
#114075=DIRECTION('center_axis',(0.978687289329817,-0.205356249870933,1.85257154385723E-5));
#114076=DIRECTION('ref_axis',(0.17767446928848,0.846806623514623,0.501348506864058));
#114077=DIRECTION('center_axis',(-1.4081690688991E-16,0.,-1.));
#114078=DIRECTION('ref_axis',(-1.,0.,1.40816906889911E-16));
#114079=DIRECTION('center_axis',(-1.4081690688991E-16,0.,-1.));
#114080=DIRECTION('ref_axis',(-1.,0.,1.4081690688991E-16));
#114081=DIRECTION('',(0.20791169081777,0.978147600733803,-2.92774812072098E-17));
#114082=DIRECTION('center_axis',(-1.4081690688991E-16,0.,-1.));
#114083=DIRECTION('ref_axis',(-1.,0.,1.4081690688991E-16));
#114084=DIRECTION('center_axis',(-1.4081690688991E-16,0.,-1.));
#114085=DIRECTION('ref_axis',(-1.,0.,1.4081690688991E-16));
#114086=DIRECTION('center_axis',(-1.4081690688991E-16,0.,-1.));
#114087=DIRECTION('ref_axis',(-1.,0.,1.4081690688991E-16));
#114088=DIRECTION('',(-0.104528463267664,-0.994521895368272,1.4719374879308E-17));
#114089=DIRECTION('center_axis',(1.4081690688991E-16,0.,1.));
#114090=DIRECTION('ref_axis',(1.,0.,-1.4081690688991E-16));
#114091=DIRECTION('',(0.103961598321227,0.489077884775272,0.866022406579785));
#114092=DIRECTION('center_axis',(1.4081690688991E-16,0.,1.));
#114093=DIRECTION('ref_axis',(-1.,3.19744231092045E-14,1.40816906889911E-16));
#114094=DIRECTION('',(-0.0522600224406464,-0.497266609935041,-0.866022406579769));
#114095=DIRECTION('center_axis',(-1.4081690688991E-16,0.,-1.));
#114096=DIRECTION('ref_axis',(-1.,0.,1.40816906889911E-16));
#114097=DIRECTION('center_axis',(-1.4081690688991E-16,0.,-1.));
#114098=DIRECTION('ref_axis',(-1.,0.,1.4081690688991E-16));
#114099=DIRECTION('',(0.20791169081777,0.978147600733803,-2.92774812072098E-17));
#114100=DIRECTION('center_axis',(1.4081690688991E-16,0.,1.));
#114101=DIRECTION('ref_axis',(-1.,3.19744231092045E-14,1.4081690688991E-16));
#114102=DIRECTION('',(-0.104528463267664,-0.994521895368272,1.4719374879308E-17));
#114103=DIRECTION('center_axis',(-1.4081690688991E-16,0.,-1.));
#114104=DIRECTION('ref_axis',(-1.,0.,1.4081690688991E-16));
#114105=DIRECTION('center_axis',(-1.4081690688991E-16,0.,-1.));
#114106=DIRECTION('ref_axis',(1.,-2.30926389122033E-14,-1.4081690688991E-16));
#114107=DIRECTION('',(0.103952356682314,0.489079645219224,-0.866022521746652));
#114108=DIRECTION('center_axis',(-1.4081690688991E-16,0.,-1.));
#114109=DIRECTION('ref_axis',(-1.,0.,1.4081690688991E-16));
#114110=DIRECTION('center_axis',(-1.4081690688991E-16,0.,-1.));
#114111=DIRECTION('ref_axis',(-1.,0.,1.4081690688991E-16));
#114112=DIRECTION('center_axis',(-1.4081690688991E-16,0.,-1.));
#114113=DIRECTION('ref_axis',(-1.,0.,1.4081690688991E-16));
#114114=DIRECTION('',(-0.0522693557686642,-0.497265428393217,0.866022521746657));
#114115=DIRECTION('center_axis',(-1.4081690688991E-16,0.,-1.));
#114116=DIRECTION('ref_axis',(-1.,0.,1.40816906889911E-16));
#114117=DIRECTION('',(0.20791169081777,0.978147600733803,-2.92774812072098E-17));
#114118=DIRECTION('center_axis',(1.4081690688991E-16,0.,1.));
#114119=DIRECTION('ref_axis',(-1.,-1.06581410364015E-14,1.4081690688991E-16));
#114120=DIRECTION('',(-0.104528463267664,-0.994521895368272,1.4719374879308E-17));
#114121=DIRECTION('center_axis',(-1.4081690688991E-16,0.,-1.));
#114122=DIRECTION('ref_axis',(-1.,0.,1.17174841180864E-16));
#114123=DIRECTION('center_axis',(0.978369559222101,-0.206864703431254,7.86457189883735E-6));
#114124=DIRECTION('ref_axis',(7.99745522015369E-6,-1.93871454059186E-7,
-0.999999999968002));
#114125=DIRECTION('center_axis',(-0.994409453539563,0.105592796389223,7.86457226736407E-6));
#114126=DIRECTION('ref_axis',(-0.0895515687886208,-0.843303350210948,-0.52992450033046));
#114127=DIRECTION('center_axis',(-1.4081690688991E-16,0.,-1.));
#114128=DIRECTION('ref_axis',(-1.,0.,1.13676889660403E-16));
#114129=DIRECTION('center_axis',(0.978360123517394,-0.206909324622083,-9.77058422961358E-6));
#114130=DIRECTION('ref_axis',(0.180976161286691,0.855713599898502,0.484769908301536));
#114131=DIRECTION('center_axis',(-0.994414268361316,0.105547443284838,-9.77051740477596E-6));
#114132=DIRECTION('ref_axis',(0.0923122812912943,0.8697641849412,0.484756336024984));
#114133=DIRECTION('center_axis',(-1.4081690688991E-16,0.,-1.));
#114134=DIRECTION('ref_axis',(-1.,0.,1.15974593313694E-16));
#114135=DIRECTION('center_axis',(-0.977604079204545,0.210452521944402,1.81624797242626E-5));
#114136=DIRECTION('ref_axis',(0.182084057577939,0.845868804766277,-0.50134953984144));
#114137=DIRECTION('center_axis',(0.994790133859855,-0.101944049587677,1.81316451691771E-5));
#114138=DIRECTION('ref_axis',(0.0883925913421295,0.862463698454322,-0.498340364253505));
#114139=DIRECTION('center_axis',(-1.4081690688991E-16,0.,-1.));
#114140=DIRECTION('ref_axis',(-1.,0.,1.16261524579732E-16));
#114141=DIRECTION('center_axis',(-0.977601235480913,0.210465731282227,1.84940584797882E-5));
#114142=DIRECTION('ref_axis',(0.18247901859632,0.847560772124576,0.498339387694488));
#114143=DIRECTION('center_axis',(0.99479151117881,-0.101930608471533,1.85257109318316E-5));
#114144=DIRECTION('ref_axis',(0.0881857549144228,0.860739767464254,0.50134850686499));
#114145=DIRECTION('center_axis',(-1.4081690688991E-16,0.,-1.));
#114146=DIRECTION('ref_axis',(-1.,0.,1.40816906889911E-16));
#114147=DIRECTION('center_axis',(-1.4081690688991E-16,0.,-1.));
#114148=DIRECTION('ref_axis',(-1.,0.,1.4081690688991E-16));
#114149=DIRECTION('',(0.104528463267664,0.994521895368272,-1.4719374879308E-17));
#114150=DIRECTION('center_axis',(-1.4081690688991E-16,0.,-1.));
#114151=DIRECTION('ref_axis',(-1.,0.,1.4081690688991E-16));
#114152=DIRECTION('center_axis',(-1.4081690688991E-16,0.,-1.));
#114153=DIRECTION('ref_axis',(-1.,0.,1.4081690688991E-16));
#114154=DIRECTION('center_axis',(-1.4081690688991E-16,0.,-1.));
#114155=DIRECTION('ref_axis',(-1.,0.,1.4081690688991E-16));
#114156=DIRECTION('',(-1.04744440165294E-14,-1.,1.4749788077992E-30));
#114157=DIRECTION('center_axis',(1.4081690688991E-16,0.,1.));
#114158=DIRECTION('ref_axis',(1.,0.,-1.4081690688991E-16));
#114159=DIRECTION('',(0.0522695260941979,0.497265611060806,0.866022406579767));
#114160=DIRECTION('center_axis',(1.4081690688991E-16,0.,1.));
#114161=DIRECTION('ref_axis',(-1.,-1.06581410364015E-14,1.40816906889911E-16));
#114162=DIRECTION('',(4.7780011601864E-6,-0.500005191252011,-0.866022406579767));
#114163=DIRECTION('center_axis',(-1.4081690688991E-16,0.,-1.));
#114164=DIRECTION('ref_axis',(-1.,0.,1.40816906889911E-16));
#114165=DIRECTION('center_axis',(-1.4081690688991E-16,0.,-1.));
#114166=DIRECTION('ref_axis',(-1.,0.,1.4081690688991E-16));
#114167=DIRECTION('',(0.104528463267664,0.994521895368272,-1.4719374879308E-17));
#114168=DIRECTION('center_axis',(1.4081690688991E-16,0.,1.));
#114169=DIRECTION('ref_axis',(-1.,-1.06581410364015E-14,1.4081690688991E-16));
#114170=DIRECTION('',(-1.04744440165294E-14,-1.,1.4749788077992E-30));
#114171=DIRECTION('center_axis',(-1.4081690688991E-16,0.,-1.));
#114172=DIRECTION('ref_axis',(-1.,0.,1.4081690688991E-16));
#114173=DIRECTION('center_axis',(-1.4081690688991E-16,0.,-1.));
#114174=DIRECTION('ref_axis',(1.,2.30926389122033E-14,-1.4081690688991E-16));
#114175=DIRECTION('',(0.0522601510654366,0.497266395846486,-0.866022521746671));
#114176=DIRECTION('center_axis',(-1.4081690688991E-16,0.,-1.));
#114177=DIRECTION('ref_axis',(-1.,0.,1.4081690688991E-16));
#114178=DIRECTION('center_axis',(-1.4081690688991E-16,0.,-1.));
#114179=DIRECTION('ref_axis',(-1.,0.,1.4081690688991E-16));
#114180=DIRECTION('center_axis',(-1.4081690688991E-16,0.,-1.));
#114181=DIRECTION('ref_axis',(-1.,0.,1.4081690688991E-16));
#114182=DIRECTION('',(-4.62770265767274E-6,-0.500004991781207,0.866022521746669));
#114183=DIRECTION('center_axis',(-1.4081690688991E-16,0.,-1.));
#114184=DIRECTION('ref_axis',(-1.,0.,1.40816906889911E-16));
#114185=DIRECTION('',(0.104528463267664,0.994521895368272,-1.4719374879308E-17));
#114186=DIRECTION('center_axis',(1.4081690688991E-16,0.,1.));
#114187=DIRECTION('ref_axis',(-1.,3.28626015289046E-14,1.4081690688991E-16));
#114188=DIRECTION('',(-1.04744440165294E-14,-1.,1.4749788077992E-30));
#114189=DIRECTION('center_axis',(-1.4081690688991E-16,0.,-1.));
#114190=DIRECTION('ref_axis',(-1.,0.,1.17174841180864E-16));
#114191=DIRECTION('center_axis',(0.994633197962181,-0.10346401040784,7.86457202285898E-6));
#114192=DIRECTION('ref_axis',(7.9739095298375E-6,6.43152272453734E-7,-0.999999999968002));
#114193=DIRECTION('center_axis',(-0.999999427244995,0.00107025596491883,
7.86457225228283E-6));
#114194=DIRECTION('ref_axis',(-0.000911792658831313,-0.848044334090885,
-0.529924500330466));
#114195=DIRECTION('center_axis',(-1.4081690688991E-16,0.,-1.));
#114196=DIRECTION('ref_axis',(-1.,0.,1.13676889660403E-16));
#114197=DIRECTION('center_axis',(0.994628478131884,-0.103509373457613,-9.77058644365307E-6));
#114198=DIRECTION('ref_axis',(0.0905383273445195,0.869943071289731,0.484769908303565));
#114199=DIRECTION('center_axis',(-0.999999475000345,0.00102464802306588,
-9.77051628361053E-6));
#114200=DIRECTION('ref_axis',(0.000891471298449509,0.874648786634599,0.484756336026202));
#114201=DIRECTION('center_axis',(-1.4081690688991E-16,0.,-1.));
#114202=DIRECTION('ref_axis',(-1.,0.,1.15974593313694E-16));
#114203=DIRECTION('center_axis',(-0.994246940479911,0.107112188925725,1.81624797550156E-5));
#114204=DIRECTION('ref_axis',(0.0926692157708285,0.860268013676602,-0.501349539835565));
#114205=DIRECTION('center_axis',(0.999996624262643,0.00259829454877897,
1.81316452302667E-5));
#114206=DIRECTION('ref_axis',(0.00224363754547992,-0.866978573809519,0.49834036425497));
#114207=DIRECTION('center_axis',(-1.4081690688991E-16,0.,-1.));
#114208=DIRECTION('ref_axis',(-1.,0.,1.16261524579732E-16));
#114209=DIRECTION('center_axis',(-0.994245493086384,0.107125623150498,1.84940602737029E-5));
#114210=DIRECTION('ref_axis',(0.0928851544029117,0.861991996922407,0.498339387700057));
#114211=DIRECTION('center_axis',(0.999996589057286,0.00261180600211936,
1.85257108473802E-5));
#114212=DIRECTION('ref_axis',(0.00226914104442804,-0.865242466405379,-0.501348506856913));
#114213=DIRECTION('center_axis',(-1.4081690688991E-16,0.,-1.));
#114214=DIRECTION('ref_axis',(-1.,0.,1.40816906889911E-16));
#114215=DIRECTION('center_axis',(-1.4081690688991E-16,0.,-1.));
#114216=DIRECTION('ref_axis',(-1.,0.,1.4081690688991E-16));
#114217=DIRECTION('',(1.04744440165294E-14,1.,-1.4749788077992E-30));
#114218=DIRECTION('center_axis',(-1.4081690688991E-16,0.,-1.));
#114219=DIRECTION('ref_axis',(-1.,0.,1.4081690688991E-16));
#114220=DIRECTION('center_axis',(-1.4081690688991E-16,0.,-1.));
#114221=DIRECTION('ref_axis',(-1.,0.,1.4081690688991E-16));
#114222=DIRECTION('center_axis',(-1.4081690688991E-16,0.,-1.));
#114223=DIRECTION('ref_axis',(-1.,0.,1.4081690688991E-16));
#114224=DIRECTION('',(0.104528463267644,-0.994521895368274,-1.47193748793052E-17));
#114225=DIRECTION('center_axis',(1.4081690688991E-16,0.,1.));
#114226=DIRECTION('ref_axis',(1.,0.,-1.4081690688991E-16));
#114227=DIRECTION('',(4.77800117084857E-6,0.500005191252011,0.866022406579767));
#114228=DIRECTION('center_axis',(1.4081690688991E-16,0.,1.));
#114229=DIRECTION('ref_axis',(-1.,-1.15463194561016E-14,1.40816906889911E-16));
#114230=DIRECTION('',(0.0522695260941891,-0.497265611060765,-0.866022406579791));
#114231=DIRECTION('center_axis',(-1.4081690688991E-16,0.,-1.));
#114232=DIRECTION('ref_axis',(-1.,0.,1.40816906889911E-16));
#114233=DIRECTION('center_axis',(-1.4081690688991E-16,0.,-1.));
#114234=DIRECTION('ref_axis',(-1.,0.,1.4081690688991E-16));
#114235=DIRECTION('',(1.04744440165294E-14,1.,-1.4749788077992E-30));
#114236=DIRECTION('center_axis',(1.4081690688991E-16,0.,1.));
#114237=DIRECTION('ref_axis',(-1.,-1.06581410364015E-14,1.4081690688991E-16));
#114238=DIRECTION('',(0.104528463267644,-0.994521895368274,-1.47193748793052E-17));
#114239=DIRECTION('center_axis',(-1.4081690688991E-16,0.,-1.));
#114240=DIRECTION('ref_axis',(-1.,0.,1.4081690688991E-16));
#114241=DIRECTION('center_axis',(-1.4081690688991E-16,0.,-1.));
#114242=DIRECTION('ref_axis',(1.,2.1316282072803E-14,-1.4081690688991E-16));
#114243=DIRECTION('',(-4.62770264722375E-6,0.500004991781227,-0.866022521746657));
#114244=DIRECTION('center_axis',(-1.4081690688991E-16,0.,-1.));
#114245=DIRECTION('ref_axis',(-1.,0.,1.4081690688991E-16));
#114246=DIRECTION('center_axis',(-1.4081690688991E-16,0.,-1.));
#114247=DIRECTION('ref_axis',(-1.,0.,1.4081690688991E-16));
#114248=DIRECTION('center_axis',(-1.4081690688991E-16,0.,-1.));
#114249=DIRECTION('ref_axis',(-1.,0.,1.4081690688991E-16));
#114250=DIRECTION('',(0.0522601510654256,-0.497266395846507,0.86602252174666));
#114251=DIRECTION('center_axis',(-1.4081690688991E-16,0.,-1.));
#114252=DIRECTION('ref_axis',(-1.,0.,1.40816906889911E-16));
#114253=DIRECTION('',(1.04744440165294E-14,1.,-1.4749788077992E-30));
#114254=DIRECTION('center_axis',(1.4081690688991E-16,0.,1.));
#114255=DIRECTION('ref_axis',(-1.,3.37507799486048E-14,1.4081690688991E-16));
#114256=DIRECTION('',(0.104528463267644,-0.994521895368274,-1.47193748793052E-17));
#114257=DIRECTION('center_axis',(-1.4081690688991E-16,0.,-1.));
#114258=DIRECTION('ref_axis',(-1.,0.,1.17174841180864E-16));
#114259=DIRECTION('center_axis',(0.999999427244995,0.00107025596477238,
7.86457202530897E-6));
#114260=DIRECTION('ref_axis',(7.86299990295297E-6,1.47312952164186E-6,-0.999999999968002));
#114261=DIRECTION('center_axis',(-0.994633197962196,-0.103464010407698,
7.86457224226079E-6));
#114262=DIRECTION('ref_axis',(0.0877379732621283,-0.843493966781848,-0.529924500330449));
#114263=DIRECTION('center_axis',(-1.4081690688991E-16,0.,-1.));
#114264=DIRECTION('ref_axis',(-1.,0.,1.13676889660403E-16));
#114265=DIRECTION('center_axis',(0.999999475000305,0.00102464806172845,
-9.77058609196671E-6));
#114266=DIRECTION('ref_axis',(0.000891463458114906,-0.874641264346845,-0.48476990830151));
#114267=DIRECTION('center_axis',(-0.994628478127934,-0.103509373495574,
-9.77051754500418E-6));
#114268=DIRECTION('ref_axis',(0.0905391058403081,-0.869950553189016,-0.484756336028486));
#114269=DIRECTION('center_axis',(-1.4081690688991E-16,0.,-1.));
#114270=DIRECTION('ref_axis',(-1.,0.,1.15974593313694E-16));
#114271=DIRECTION('center_axis',(-0.999996624215829,0.00259831235054303,
1.81624797937814E-5));
#114272=DIRECTION('ref_axis',(0.0022390706427464,0.86524194619802,-0.501349539844328));
#114273=DIRECTION('center_axis',(0.994246942387258,0.107112171226391,1.81316452305702E-5));
#114274=DIRECTION('ref_axis',(0.0928552846705921,-0.861994650484445,0.498340364254134));
#114275=DIRECTION('center_axis',(-1.4081690688991E-16,0.,-1.));
#114276=DIRECTION('ref_axis',(-1.,0.,1.16261524579732E-16));
#114277=DIRECTION('center_axis',(-0.999996589010146,0.0026118242750869,
1.84940601186701E-5));
#114278=DIRECTION('ref_axis',(0.00227362102102081,0.866979057023919,0.498339387696144));
#114279=DIRECTION('center_axis',(0.994245495043238,0.107125604983238,1.85257097596897E-5));
#114280=DIRECTION('ref_axis',(0.0926991758193815,-0.860265387814003,-0.501348506860876));
#114281=DIRECTION('center_axis',(-1.4081690688991E-16,0.,-1.));
#114282=DIRECTION('ref_axis',(-1.,0.,1.40816906889911E-16));
#114283=DIRECTION('center_axis',(-1.4081690688991E-16,0.,-1.));
#114284=DIRECTION('ref_axis',(-1.,0.,1.4081690688991E-16));
#114285=DIRECTION('',(-0.104528463267644,0.994521895368274,1.47193748793052E-17));
#114286=DIRECTION('center_axis',(-1.4081690688991E-16,0.,-1.));
#114287=DIRECTION('ref_axis',(-1.,0.,1.4081690688991E-16));
#114288=DIRECTION('center_axis',(-1.4081690688991E-16,0.,-1.));
#114289=DIRECTION('ref_axis',(-1.,0.,1.4081690688991E-16));
#114290=DIRECTION('center_axis',(-1.4081690688991E-16,0.,-1.));
#114291=DIRECTION('ref_axis',(-1.,0.,1.4081690688991E-16));
#114292=DIRECTION('',(0.207911690817749,-0.978147600733808,-2.92774812072069E-17));
#114293=DIRECTION('center_axis',(1.4081690688991E-16,0.,1.));
#114294=DIRECTION('ref_axis',(1.,0.,-1.4081690688991E-16));
#114295=DIRECTION('',(-0.0522600224406444,0.497266609935,0.866022406579793));
#114296=DIRECTION('center_axis',(1.4081690688991E-16,0.,1.));
#114297=DIRECTION('ref_axis',(-1.,3.37507799486048E-14,1.40816906889911E-16));
#114298=DIRECTION('',(0.103961598321227,-0.489077884775272,-0.866022406579785));
#114299=DIRECTION('center_axis',(-1.4081690688991E-16,0.,-1.));
#114300=DIRECTION('ref_axis',(-1.,0.,1.40816906889911E-16));
#114301=DIRECTION('center_axis',(-1.4081690688991E-16,0.,-1.));
#114302=DIRECTION('ref_axis',(-1.,0.,1.4081690688991E-16));
#114303=DIRECTION('',(-0.104528463267644,0.994521895368274,1.47193748793052E-17));
#114304=DIRECTION('center_axis',(1.4081690688991E-16,0.,1.));
#114305=DIRECTION('ref_axis',(-1.,3.46389583683049E-14,1.4081690688991E-16));
#114306=DIRECTION('',(0.207911690817749,-0.978147600733808,-2.92774812072069E-17));
#114307=DIRECTION('center_axis',(-1.4081690688991E-16,0.,-1.));
#114308=DIRECTION('ref_axis',(-1.,0.,1.4081690688991E-16));
#114309=DIRECTION('center_axis',(-1.4081690688991E-16,0.,-1.));
#114310=DIRECTION('ref_axis',(1.,-2.1316282072803E-14,-1.4081690688991E-16));
#114311=DIRECTION('',(-0.0522693557686574,0.497265428393217,-0.866022521746658));
#114312=DIRECTION('center_axis',(-1.4081690688991E-16,0.,-1.));
#114313=DIRECTION('ref_axis',(-1.,0.,1.4081690688991E-16));
#114314=DIRECTION('center_axis',(-1.4081690688991E-16,0.,-1.));
#114315=DIRECTION('ref_axis',(-1.,0.,1.4081690688991E-16));
#114316=DIRECTION('center_axis',(-1.4081690688991E-16,0.,-1.));
#114317=DIRECTION('ref_axis',(-1.,0.,1.4081690688991E-16));
#114318=DIRECTION('',(0.103952356682308,-0.489079645219204,0.866022521746664));
#114319=DIRECTION('center_axis',(-1.4081690688991E-16,0.,-1.));
#114320=DIRECTION('ref_axis',(-1.,0.,1.40816906889911E-16));
#114321=DIRECTION('',(-0.104528463267644,0.994521895368274,1.47193748793052E-17));
#114322=DIRECTION('center_axis',(1.4081690688991E-16,0.,1.));
#114323=DIRECTION('ref_axis',(-1.,-1.06581410364015E-14,1.4081690688991E-16));
#114324=DIRECTION('',(0.207911690817749,-0.978147600733808,-2.92774812072069E-17));
#114325=DIRECTION('center_axis',(-1.4081690688991E-16,0.,-1.));
#114326=DIRECTION('ref_axis',(-1.,0.,1.17174841180864E-16));
#114327=DIRECTION('center_axis',(0.994409453539581,0.105592796389056,7.86457200107375E-6));
#114328=DIRECTION('ref_axis',(7.66594157259133E-6,2.28696690243279E-6,-0.999999999968002));
#114329=DIRECTION('center_axis',(-0.978369559222145,-0.206864703431043,
7.86457225237907E-6));
#114330=DIRECTION('ref_axis',(0.175426463587655,-0.82970210306027,-0.529924500330466));
#114331=DIRECTION('center_axis',(-1.4081690688991E-16,0.,-1.));
#114332=DIRECTION('ref_axis',(-1.,0.,1.13676889660403E-16));
#114333=DIRECTION('center_axis',(0.994414268357315,0.105547443322528,-9.77058581902262E-6));
#114334=DIRECTION('ref_axis',(0.0923114872006239,-0.869756704679759,-0.484769908302295));
#114335=DIRECTION('center_axis',(-0.978360123509492,-0.206909324659449,
-9.77051516979182E-6));
#114336=DIRECTION('ref_axis',(0.180977717589048,-0.85572095943558,-0.484756336027606));
#114337=DIRECTION('center_axis',(-1.4081690688991E-16,0.,-1.));
#114338=DIRECTION('ref_axis',(-1.,0.,1.15974593313694E-16));
#114339=DIRECTION('center_axis',(-0.994790135674097,-0.101944031878453,
1.81624797954842E-5));
#114340=DIRECTION('ref_axis',(0.0882156062112984,-0.860736106898752,0.501349539843762));
#114341=DIRECTION('center_axis',(0.97760408295153,0.210452504541384,1.81316452299228E-5));
#114342=DIRECTION('ref_axis',(0.182449589866239,-0.847566533387013,0.498340364249137));
#114343=DIRECTION('center_axis',(-1.4081690688991E-16,0.,-1.));
#114344=DIRECTION('ref_axis',(-1.,0.,1.16261524579732E-16));
#114345=DIRECTION('center_axis',(-0.994791513041914,-0.101930590294321,
1.84940611814327E-5));
#114346=DIRECTION('ref_axis',(0.0883628226288923,-0.862467313148419,-0.498339387694373));
#114347=DIRECTION('center_axis',(0.977601239326121,0.210465713418671,1.85257086791728E-5));
#114348=DIRECTION('ref_axis',(0.182113579025865,-0.84586306161554,-0.501348506858029));
#114349=DIRECTION('center_axis',(-1.4081690688991E-16,0.,-1.));
#114350=DIRECTION('ref_axis',(-1.,0.,1.40816906889911E-16));
#114351=DIRECTION('center_axis',(-1.4081690688991E-16,0.,-1.));
#114352=DIRECTION('ref_axis',(-1.,0.,1.4081690688991E-16));
#114353=DIRECTION('',(-0.207911690817749,0.978147600733808,2.92774812072069E-17));
#114354=DIRECTION('center_axis',(-1.4081690688991E-16,0.,-1.));
#114355=DIRECTION('ref_axis',(-1.,0.,1.4081690688991E-16));
#114356=DIRECTION('center_axis',(-1.4081690688991E-16,0.,-1.));
#114357=DIRECTION('ref_axis',(-1.,0.,1.4081690688991E-16));
#114358=DIRECTION('center_axis',(-1.4081690688991E-16,0.,-1.));
#114359=DIRECTION('ref_axis',(-1.,0.,1.4081690688991E-16));
#114360=DIRECTION('',(0.309016994374938,-0.951056516295157,-4.35148173242957E-17));
#114361=DIRECTION('center_axis',(1.4081690688991E-16,0.,1.));
#114362=DIRECTION('ref_axis',(1.,0.,-1.4081690688991E-16));
#114363=DIRECTION('',(-0.103952251140481,0.489079871579878,0.866022406579781));
#114364=DIRECTION('center_axis',(1.4081690688991E-16,0.,1.));
#114365=DIRECTION('ref_axis',(-1.,3.46389583683049E-14,1.40816906889911E-16));
#114366=DIRECTION('',(0.154514645521709,-0.475531718838051,-0.866022406579778));
#114367=DIRECTION('center_axis',(-1.4081690688991E-16,0.,-1.));
#114368=DIRECTION('ref_axis',(-1.,0.,1.40816906889911E-16));
#114369=DIRECTION('center_axis',(-1.4081690688991E-16,0.,-1.));
#114370=DIRECTION('ref_axis',(-1.,0.,1.4081690688991E-16));
#114371=DIRECTION('',(-0.207911690817749,0.978147600733808,2.92774812072069E-17));
#114372=DIRECTION('center_axis',(1.4081690688991E-16,0.,1.));
#114373=DIRECTION('ref_axis',(-1.,3.5527136788005E-14,1.4081690688991E-16));
#114374=DIRECTION('',(0.309016994374938,-0.951056516295157,-4.35148173242957E-17));
#114375=DIRECTION('center_axis',(-1.4081690688991E-16,0.,-1.));
#114376=DIRECTION('ref_axis',(-1.,0.,1.4081690688991E-16));
#114377=DIRECTION('center_axis',(-1.4081690688991E-16,0.,-1.));
#114378=DIRECTION('ref_axis',(1.,-2.1316282072803E-14,-1.4081690688991E-16));
#114379=DIRECTION('',(-0.103961409834804,0.489077720912242,-0.866022521746662));
#114380=DIRECTION('center_axis',(-1.4081690688991E-16,0.,-1.));
#114381=DIRECTION('ref_axis',(-1.,0.,1.4081690688991E-16));
#114382=DIRECTION('center_axis',(-1.4081690688991E-16,0.,-1.));
#114383=DIRECTION('ref_axis',(-1.,0.,1.4081690688991E-16));
#114384=DIRECTION('center_axis',(-1.4081690688991E-16,0.,-1.));
#114385=DIRECTION('ref_axis',(-1.,0.,1.4081690688991E-16));
#114386=DIRECTION('',(0.154505638525955,-0.475534435652359,0.86602252174668));
#114387=DIRECTION('center_axis',(-1.4081690688991E-16,0.,-1.));
#114388=DIRECTION('ref_axis',(-1.,0.,1.40816906889911E-16));
#114389=DIRECTION('',(-0.207911690817749,0.978147600733808,2.92774812072069E-17));
#114390=DIRECTION('center_axis',(1.4081690688991E-16,0.,1.));
#114391=DIRECTION('ref_axis',(-1.,0.,1.4081690688991E-16));
#114392=DIRECTION('',(0.309016994374938,-0.951056516295157,-4.35148173242957E-17));
#114393=DIRECTION('center_axis',(-1.4081690688991E-16,0.,-1.));
#114394=DIRECTION('ref_axis',(-1.,0.,1.17174841180864E-16));
#114395=DIRECTION('center_axis',(0.977924521767646,0.208958440039328,7.86457187141246E-6));
#114396=DIRECTION('ref_axis',(7.38489348936258E-6,3.07574769236174E-6,-0.999999999968002));
#114397=DIRECTION('center_axis',(-0.951386698854274,-0.307998943474349,
7.86457230114699E-6));
#114398=DIRECTION('ref_axis',(0.261192944867729,-0.80681984947127,-0.529924500330453));
#114399=DIRECTION('center_axis',(-1.4081690688991E-16,0.,-1.));
#114400=DIRECTION('ref_axis',(-1.,0.,1.13676889660403E-16));
#114401=DIRECTION('center_axis',(0.977934050896062,0.208913838705231,-9.77058216020036E-6));
#114402=DIRECTION('ref_axis',(0.182720126971813,-0.855342908547742,-0.484769908303406));
#114403=DIRECTION('center_axis',(-0.951372650642299,-0.308042333964641,
-9.77051105240763E-6));
#114404=DIRECTION('ref_axis',(0.269433499591965,-0.832115907779489,-0.48475633602661));
#114405=DIRECTION('center_axis',(-1.4081690688991E-16,0.,-1.));
#114406=DIRECTION('ref_axis',(-1.,0.,1.15974593313694E-16));
#114407=DIRECTION('center_axis',(-0.978684518232684,-0.205369455961164,
1.81624797100977E-5));
#114408=DIRECTION('ref_axis',(0.177703774423794,-0.846799862692929,0.501349539840991));
#114409=DIRECTION('center_axis',(0.950250388606192,0.311487076176564,1.81316452056593E-5));
#114410=DIRECTION('ref_axis',(0.270044939174703,-0.823852299981494,0.498340364250513));
#114411=DIRECTION('center_axis',(-1.4081690688991E-16,0.,-1.));
#114412=DIRECTION('ref_axis',(-1.,0.,1.16261524579732E-16));
#114413=DIRECTION('center_axis',(-0.978687293084006,-0.205356231982065,
1.84940551457799E-5));
#114414=DIRECTION('ref_axis',(0.178031144703053,-0.848506196906717,-0.498339387693387));
#114415=DIRECTION('center_axis',(0.9502461798562,0.311499915450223,1.85257163965025E-5));
#114416=DIRECTION('ref_axis',(0.269532707749906,-0.822193282701928,-0.501348506862074));
#114417=DIRECTION('center_axis',(-1.4081690688991E-16,0.,-1.));
#114418=DIRECTION('ref_axis',(-1.,0.,1.40816906889911E-16));
#114419=DIRECTION('center_axis',(-1.4081690688991E-16,0.,-1.));
#114420=DIRECTION('ref_axis',(-1.,0.,1.4081690688991E-16));
#114421=DIRECTION('',(-0.309016994374938,0.951056516295157,4.35148173242957E-17));
#114422=DIRECTION('center_axis',(-1.4081690688991E-16,0.,-1.));
#114423=DIRECTION('ref_axis',(-1.,0.,1.4081690688991E-16));
#114424=DIRECTION('center_axis',(-1.4081690688991E-16,0.,-1.));
#114425=DIRECTION('ref_axis',(-1.,0.,1.4081690688991E-16));
#114426=DIRECTION('center_axis',(-1.4081690688991E-16,0.,-1.));
#114427=DIRECTION('ref_axis',(-1.,0.,1.4081690688991E-16));
#114428=DIRECTION('',(0.406736643075792,-0.913545457642605,-5.72753959967185E-17));
#114429=DIRECTION('center_axis',(1.4081690688991E-16,0.,1.));
#114430=DIRECTION('ref_axis',(1.,0.,-1.4081690688991E-16));
#114431=DIRECTION('',(-0.154505557223403,0.475534671805168,0.866022406579782));
#114432=DIRECTION('center_axis',(1.4081690688991E-16,0.,1.));
#114433=DIRECTION('ref_axis',(-1.,0.,1.40816906889911E-16));
#114434=DIRECTION('',(0.203374797931583,-0.456775527877804,-0.866022406579785));
#114435=DIRECTION('center_axis',(-1.4081690688991E-16,0.,-1.));
#114436=DIRECTION('ref_axis',(-1.,0.,1.40816906889911E-16));
#114437=DIRECTION('center_axis',(-1.4081690688991E-16,0.,-1.));
#114438=DIRECTION('ref_axis',(-1.,0.,1.4081690688991E-16));
#114439=DIRECTION('',(-0.309016994374938,0.951056516295157,4.35148173242957E-17));
#114440=DIRECTION('center_axis',(1.4081690688991E-16,0.,1.));
#114441=DIRECTION('ref_axis',(-1.,3.5527136788005E-14,1.4081690688991E-16));
#114442=DIRECTION('',(0.406736643075792,-0.913545457642605,-5.72753959967185E-17));
#114443=DIRECTION('center_axis',(-1.4081690688991E-16,0.,-1.));
#114444=DIRECTION('ref_axis',(-1.,0.,1.4081690688991E-16));
#114445=DIRECTION('center_axis',(-1.4081690688991E-16,0.,-1.));
#114446=DIRECTION('ref_axis',(1.,-1.95399252334028E-14,-1.4081690688991E-16));
#114447=DIRECTION('',(-0.154514440939472,0.475531575574881,-0.866022521746654));
#114448=DIRECTION('center_axis',(-1.4081690688991E-16,0.,-1.));
#114449=DIRECTION('ref_axis',(-1.,0.,1.4081690688991E-16));
#114450=DIRECTION('center_axis',(-1.4081690688991E-16,0.,-1.));
#114451=DIRECTION('ref_axis',(-1.,0.,1.4081690688991E-16));
#114452=DIRECTION('center_axis',(-1.4081690688991E-16,0.,-1.));
#114453=DIRECTION('ref_axis',(-1.,0.,1.4081690688991E-16));
#114454=DIRECTION('',(0.2033661242615,-0.456779171296606,0.866022521746659));
#114455=DIRECTION('center_axis',(-1.4081690688991E-16,0.,-1.));
#114456=DIRECTION('ref_axis',(-1.,0.,1.40816906889911E-16));
#114457=DIRECTION('',(-0.309016994374938,0.951056516295157,4.35148173242957E-17));
#114458=DIRECTION('center_axis',(1.4081690688991E-16,0.,1.));
#114459=DIRECTION('ref_axis',(-1.,0.,1.4081690688991E-16));
#114460=DIRECTION('',(0.406736643075792,-0.913545457642605,-5.72753959967185E-17));
#114461=DIRECTION('center_axis',(-1.4081690688991E-16,0.,-1.));
#114462=DIRECTION('ref_axis',(-1.,0.,1.17174841180864E-16));
#114463=DIRECTION('center_axis',(0.950725244291326,0.310034691293324,7.86457201959739E-6));
#114464=DIRECTION('ref_axis',(7.02293523252021E-6,3.83083002565365E-6,-0.999999999968001));
#114465=DIRECTION('center_axis',(-0.91398024672327,-0.405758682640088,7.86457224839801E-6));
#114466=DIRECTION('ref_axis',(0.3440977415858,-0.775097908773512,-0.529924500330454));
#114467=DIRECTION('center_axis',(-1.4081690688991E-16,0.,-1.));
#114468=DIRECTION('ref_axis',(-1.,0.,1.13676889660403E-16));
#114469=DIRECTION('center_axis',(0.950739383326775,0.309991330356124,-9.77058418244769E-6));
#114470=DIRECTION('ref_axis',(0.271126846795278,-0.831557796518166,-0.484769908303621));
#114471=DIRECTION('center_axis',(-0.913961739929031,-0.4058003669915,-9.77051737432389E-6));
#114472=DIRECTION('ref_axis',(0.354937311790693,-0.799394020105817,-0.48475633602652));
#114473=DIRECTION('center_axis',(-1.4081690688991E-16,0.,-1.));
#114474=DIRECTION('ref_axis',(-1.,0.,1.15974593313694E-16));
#114475=DIRECTION('center_axis',(-0.95185622840661,-0.306544809307982,1.81624796416327E-5));
#114476=DIRECTION('ref_axis',(0.265244982895815,-0.823585901983176,0.501349539845363));
#114477=DIRECTION('center_axis',(0.912485552150587,0.409108930222359,1.81316451411862E-5));
#114478=DIRECTION('ref_axis',(0.354681619616753,-0.791111768370323,0.498340364261231));
#114479=DIRECTION('center_axis',(-1.4081690688991E-16,0.,-1.));
#114480=DIRECTION('ref_axis',(-1.,0.,1.16261524579732E-16));
#114481=DIRECTION('center_axis',(-0.951860370340397,-0.306531947818513,
1.84940485141779E-5));
#114482=DIRECTION('ref_axis',(0.265748920300392,-0.825248669209763,-0.498339387693458));
#114483=DIRECTION('center_axis',(0.91248002438436,0.409121259232902,1.85257051375691E-5));
#114484=DIRECTION('ref_axis',(0.353998779725107,-0.789515382130535,-0.501348506861654));
#114485=DIRECTION('center_axis',(-1.4081690688991E-16,0.,-1.));
#114486=DIRECTION('ref_axis',(-1.,0.,1.40816906889911E-16));
#114487=DIRECTION('center_axis',(-1.4081690688991E-16,0.,-1.));
#114488=DIRECTION('ref_axis',(-1.,0.,1.4081690688991E-16));
#114489=DIRECTION('',(-0.406736643075792,0.913545457642605,5.72753959967185E-17));
#114490=DIRECTION('center_axis',(-1.4081690688991E-16,0.,-1.));
#114491=DIRECTION('ref_axis',(-1.,0.,1.4081690688991E-16));
#114492=DIRECTION('center_axis',(-1.4081690688991E-16,0.,-1.));
#114493=DIRECTION('ref_axis',(-1.,0.,1.4081690688991E-16));
#114494=DIRECTION('center_axis',(-1.4081690688991E-16,0.,-1.));
#114495=DIRECTION('ref_axis',(-1.,0.,1.4081690688991E-16));
#114496=DIRECTION('',(0.499999999999992,-0.866025403784443,-7.04084534449541E-17));
#114497=DIRECTION('center_axis',(1.4081690688991E-16,0.,1.));
#114498=DIRECTION('ref_axis',(1.,0.,-1.4081690688991E-16));
#114499=DIRECTION('',(-0.203366068089009,0.456779414654112,0.866022406579797));
#114500=DIRECTION('center_axis',(1.4081690688991E-16,0.,1.));
#114501=DIRECTION('ref_axis',(-1.,0.,1.40816906889911E-16));
#114502=DIRECTION('',(0.250006733496392,-0.433014808647731,-0.866022406579779));
#114503=DIRECTION('center_axis',(-1.4081690688991E-16,0.,-1.));
#114504=DIRECTION('ref_axis',(-1.,0.,1.40816906889911E-16));
#114505=DIRECTION('center_axis',(-1.4081690688991E-16,0.,-1.));
#114506=DIRECTION('ref_axis',(-1.,0.,1.4081690688991E-16));
#114507=DIRECTION('',(-0.406736643075792,0.913545457642605,5.72753959967185E-17));
#114508=DIRECTION('center_axis',(1.4081690688991E-16,0.,1.));
#114509=DIRECTION('ref_axis',(-1.,-1.15463194561016E-14,1.4081690688991E-16));
#114510=DIRECTION('',(0.499999999999992,-0.866025403784443,-7.04084534449541E-17));
#114511=DIRECTION('center_axis',(-1.4081690688991E-16,0.,-1.));
#114512=DIRECTION('ref_axis',(-1.,0.,1.4081690688991E-16));
#114513=DIRECTION('center_axis',(-1.4081690688991E-16,0.,-1.));
#114514=DIRECTION('ref_axis',(1.,1.06581410364015E-14,-1.4081690688991E-16));
#114515=DIRECTION('',(-0.203374579494982,0.456775406784115,-0.866022521746661));
#114516=DIRECTION('center_axis',(-1.4081690688991E-16,0.,-1.));
#114517=DIRECTION('ref_axis',(-1.,0.,1.4081690688991E-16));
#114518=DIRECTION('center_axis',(-1.4081690688991E-16,0.,-1.));
#114519=DIRECTION('ref_axis',(-1.,0.,1.4081690688991E-16));
#114520=DIRECTION('center_axis',(-1.4081690688991E-16,0.,-1.));
#114521=DIRECTION('ref_axis',(-1.,0.,1.4081690688991E-16));
#114522=DIRECTION('',(0.249998488182543,-0.433019338752907,0.866022521746657));
#114523=DIRECTION('center_axis',(-1.4081690688991E-16,0.,-1.));
#114524=DIRECTION('ref_axis',(-1.,0.,1.40816906889911E-16));
#114525=DIRECTION('',(-0.406736643075792,0.913545457642605,5.72753959967185E-17));
#114526=DIRECTION('center_axis',(1.4081690688991E-16,0.,1.));
#114527=DIRECTION('ref_axis',(-1.,0.,1.4081690688991E-16));
#114528=DIRECTION('',(0.499999999999992,-0.866025403784443,-7.04084534449541E-17));
#114529=DIRECTION('center_axis',(-1.4081690688991E-16,0.,-1.));
#114530=DIRECTION('ref_axis',(-1.,0.,1.17174841180864E-16));
#114531=DIRECTION('center_axis',(0.913109622086558,0.407714137590409,7.86457186754196E-6));
#114532=DIRECTION('ref_axis',(6.58403193953515E-6,4.54394091320277E-6,-0.999999999968002));
#114533=DIRECTION('center_axis',(-0.866560035746524,-0.499072844768309,
7.86457228533342E-6));
#114534=DIRECTION('ref_axis',(0.423232531439884,-0.734883833187603,-0.529924500330456));
#114535=DIRECTION('center_axis',(-1.4081690688991E-16,0.,-1.));
#114536=DIRECTION('ref_axis',(-1.,0.,1.13676889660403E-16));
#114537=DIRECTION('center_axis',(0.913128216116848,0.40767249212548,-9.77059363821822E-6));
#114538=DIRECTION('ref_axis',(0.356563044148667,-0.79866196325611,-0.484769908302208));
#114539=DIRECTION('center_axis',(-0.866537273133093,-0.499112366281983,
-9.77051681670262E-6));
#114540=DIRECTION('ref_axis',(0.436552356525271,-0.75791380426263,-0.484756336029123));
#114541=DIRECTION('center_axis',(-1.4081690688991E-16,0.,-1.));
#114542=DIRECTION('ref_axis',(-1.,0.,1.15974593313694E-16));
#114543=DIRECTION('center_axis',(-0.914599202553385,-0.404361593575401,
1.81624795807573E-5));
#114544=DIRECTION('ref_axis',(0.349880111829649,-0.791348561787279,0.501349539845484));
#114545=DIRECTION('center_axis',(0.86472333303575,0.502248501217064,1.81316452677056E-5));
#114546=DIRECTION('ref_axis',(0.43543233401603,-0.749703650683173,0.49834036425487));
#114547=DIRECTION('center_axis',(-1.4081690688991E-16,0.,-1.));
#114548=DIRECTION('ref_axis',(-1.,0.,1.16261524579732E-16));
#114549=DIRECTION('center_axis',(-0.914604666187431,-0.404349235495936,
1.84940550607155E-5));
#114550=DIRECTION('ref_axis',(0.35055509511501,-0.792949544397653,-0.498339387695234));
#114551=DIRECTION('center_axis',(0.864716546818594,0.502260184879236,1.85257048927828E-5));
#114552=DIRECTION('ref_axis',(0.434586366991679,-0.748187385817474,-0.501348506857843));
#114553=DIRECTION('center_axis',(-1.4081690688991E-16,0.,-1.));
#114554=DIRECTION('ref_axis',(-1.,0.,1.40816906889911E-16));
#114555=DIRECTION('center_axis',(-1.4081690688991E-16,0.,-1.));
#114556=DIRECTION('ref_axis',(-1.,0.,1.4081690688991E-16));
#114557=DIRECTION('',(-0.499999999999992,0.866025403784443,7.04084534449541E-17));
#114558=DIRECTION('center_axis',(-1.4081690688991E-16,0.,-1.));
#114559=DIRECTION('ref_axis',(-1.,0.,1.4081690688991E-16));
#114560=DIRECTION('center_axis',(-1.4081690688991E-16,0.,-1.));
#114561=DIRECTION('ref_axis',(-1.,0.,1.4081690688991E-16));
#114562=DIRECTION('center_axis',(-1.4081690688991E-16,0.,-1.));
#114563=DIRECTION('ref_axis',(-1.,0.,1.4081690688991E-16));
#114564=DIRECTION('',(0.587785252292466,-0.809016994374953,-8.27701011433307E-17));
#114565=DIRECTION('center_axis',(1.4081690688991E-16,0.,1.));
#114566=DIRECTION('ref_axis',(1.,0.,-1.4081690688991E-16));
#114567=DIRECTION('',(-0.249998457755585,0.433019586648859,0.866022406579807));
#114568=DIRECTION('center_axis',(1.4081690688991E-16,0.,1.));
#114569=DIRECTION('ref_axis',(-1.,-1.24344978758018E-14,1.40816906889911E-16));
#114570=DIRECTION('',(0.29389954297172,-0.404509888559932,-0.866022406579787));
#114571=DIRECTION('center_axis',(-1.4081690688991E-16,0.,-1.));
#114572=DIRECTION('ref_axis',(-1.,0.,1.40816906889911E-16));
#114573=DIRECTION('center_axis',(-1.4081690688991E-16,0.,-1.));
#114574=DIRECTION('ref_axis',(-1.,0.,1.4081690688991E-16));
#114575=DIRECTION('',(-0.499999999999992,0.866025403784443,7.04084534449541E-17));
#114576=DIRECTION('center_axis',(1.4081690688991E-16,0.,1.));
#114577=DIRECTION('ref_axis',(-1.,3.01980662698043E-14,1.4081690688991E-16));
#114578=DIRECTION('',(0.587785252292466,-0.809016994374953,-8.27701011433307E-17));
#114579=DIRECTION('center_axis',(-1.4081690688991E-16,0.,-1.));
#114580=DIRECTION('ref_axis',(-1.,0.,1.4081690688991E-16));
#114581=DIRECTION('center_axis',(-1.4081690688991E-16,0.,-1.));
#114582=DIRECTION('ref_axis',(1.,1.95399252334028E-14,-1.4081690688991E-16));
#114583=DIRECTION('',(-0.25000650359866,0.433014711050234,-0.866022521746667));
#114584=DIRECTION('center_axis',(-1.4081690688991E-16,0.,-1.));
#114585=DIRECTION('ref_axis',(-1.,0.,1.4081690688991E-16));
#114586=DIRECTION('center_axis',(-1.4081690688991E-16,0.,-1.));
#114587=DIRECTION('ref_axis',(-1.,0.,1.4081690688991E-16));
#114588=DIRECTION('center_axis',(-1.4081690688991E-16,0.,-1.));
#114589=DIRECTION('ref_axis',(-1.,0.,1.4081690688991E-16));
#114590=DIRECTION('',(0.293891816351498,-0.404515255718706,0.866022521746661));
#114591=DIRECTION('center_axis',(-1.4081690688991E-16,0.,-1.));
#114592=DIRECTION('ref_axis',(-1.,0.,1.40816906889911E-16));
#114593=DIRECTION('',(-0.499999999999992,0.866025403784443,7.04084534449541E-17));
#114594=DIRECTION('center_axis',(1.4081690688991E-16,0.,1.));
#114595=DIRECTION('ref_axis',(-1.,-6.21724893790088E-15,1.4081690688991E-16));
#114596=DIRECTION('',(0.587785252292466,-0.809016994374953,-8.27701011433307E-17));
#114597=DIRECTION('center_axis',(-1.4081690688991E-16,0.,-1.));
#114598=DIRECTION('ref_axis',(-1.,0.,1.17174841180864E-16));
#114599=DIRECTION('center_axis',(0.865489779781645,0.500926582476583,7.86457206261499E-6));
#114600=DIRECTION('ref_axis',(6.07299293807602E-6,5.20726754909509E-6,-0.999999999968002));
#114601=DIRECTION('center_axis',(-0.809645611678775,-0.586919060371574,
7.86457229727665E-6));
#114602=DIRECTION('ref_axis',(0.497730297112456,-0.686618216540951,-0.529924500330443));
#114603=DIRECTION('center_axis',(-1.4081690688991E-16,0.,-1.));
#114604=DIRECTION('ref_axis',(-1.,0.,1.13676889660403E-16));
#114605=DIRECTION('center_axis',(0.865512625088529,0.500887108754956,-9.7705931674539E-6));
#114606=DIRECTION('ref_axis',(0.438092662174321,-0.757015822392775,-0.484769908302905));
#114607=DIRECTION('center_axis',(-0.809618842639843,-0.586955986039037,
-9.77052175743205E-6));
#114608=DIRECTION('ref_axis',(0.513384442289742,-0.7081297261801,-0.484756336023519));
#114609=DIRECTION('center_axis',(-1.4081690688991E-16,0.,-1.));
#114610=DIRECTION('ref_axis',(-1.,0.,1.15974593313694E-16));
#114611=DIRECTION('center_axis',(-0.86732163644481,-0.497748107605465,1.81624796484551E-5));
#114612=DIRECTION('ref_axis',(0.430681881041749,-0.750441041149111,0.50134953984359));
#114613=DIRECTION('center_axis',(0.807487024129162,0.589885332530207,1.81316450787733E-5));
#114614=DIRECTION('ref_axis',(0.511412360643632,-0.700081622911792,0.49834036425128));
#114615=DIRECTION('center_axis',(-1.4081690688991E-16,0.,-1.));
#114616=DIRECTION('ref_axis',(-1.,0.,1.16261524579732E-16));
#114617=DIRECTION('center_axis',(-0.867328361918051,-0.49773638833274,1.84940603276878E-5));
#114618=DIRECTION('ref_axis',(0.431520514948258,-0.751962698440682,-0.498339387699386));
#114619=DIRECTION('center_axis',(0.807479053809579,0.589896242839014,1.85256966566585E-5));
#114620=DIRECTION('ref_axis',(0.510412535074995,-0.698662091931687,-0.501348506865191));
#114621=DIRECTION('center_axis',(-1.4081690688991E-16,0.,-1.));
#114622=DIRECTION('ref_axis',(-1.,0.,1.40816906889911E-16));
#114623=DIRECTION('center_axis',(-1.4081690688991E-16,0.,-1.));
#114624=DIRECTION('ref_axis',(-1.,0.,1.4081690688991E-16));
#114625=DIRECTION('',(-0.587785252292466,0.809016994374953,8.27701011433307E-17));
#114626=DIRECTION('center_axis',(-1.4081690688991E-16,0.,-1.));
#114627=DIRECTION('ref_axis',(-1.,0.,1.4081690688991E-16));
#114628=DIRECTION('center_axis',(-1.4081690688991E-16,0.,-1.));
#114629=DIRECTION('ref_axis',(-1.,0.,1.4081690688991E-16));
#114630=DIRECTION('center_axis',(-1.4081690688991E-16,0.,-1.));
#114631=DIRECTION('ref_axis',(-1.,0.,1.4081690688991E-16));
#114632=DIRECTION('',(0.669130606358852,-0.7431448254774,-9.42249022928238E-17));
#114633=DIRECTION('center_axis',(1.4081690688991E-16,0.,1.));
#114634=DIRECTION('ref_axis',(1.,0.,-1.4081690688991E-16));
#114635=DIRECTION('',(-0.293891812003425,0.404515505437168,0.866022406579793));
#114636=DIRECTION('center_axis',(1.4081690688991E-16,0.,1.));
#114637=DIRECTION('ref_axis',(-1.,1.86517468137026E-14,1.40816906889911E-16));
#114638=DIRECTION('',(0.334572327551833,-0.371573073483921,-0.866022406579796));
#114639=DIRECTION('center_axis',(-1.4081690688991E-16,0.,-1.));
#114640=DIRECTION('ref_axis',(-1.,0.,1.40816906889911E-16));
#114641=DIRECTION('center_axis',(-1.4081690688991E-16,0.,-1.));
#114642=DIRECTION('ref_axis',(-1.,0.,1.4081690688991E-16));
#114643=DIRECTION('',(-0.587785252292466,0.809016994374953,8.27701011433307E-17));
#114644=DIRECTION('center_axis',(1.4081690688991E-16,0.,1.));
#114645=DIRECTION('ref_axis',(-1.,2.48689957516035E-14,1.4081690688991E-16));
#114646=DIRECTION('',(0.669130606358852,-0.7431448254774,-9.42249022928238E-17));
#114647=DIRECTION('center_axis',(-1.4081690688991E-16,0.,-1.));
#114648=DIRECTION('ref_axis',(-1.,0.,1.4081690688991E-16));
#114649=DIRECTION('center_axis',(-1.4081690688991E-16,0.,-1.));
#114650=DIRECTION('ref_axis',(1.,0.,-1.4081690688991E-16));
#114651=DIRECTION('',(-0.293899304131723,0.404509815527924,-0.866022521746666));
#114652=DIRECTION('center_axis',(-1.4081690688991E-16,0.,-1.));
#114653=DIRECTION('ref_axis',(-1.,0.,1.4081690688991E-16));
#114654=DIRECTION('center_axis',(-1.4081690688991E-16,0.,-1.));
#114655=DIRECTION('ref_axis',(-1.,0.,1.4081690688991E-16));
#114656=DIRECTION('center_axis',(-1.4081690688991E-16,0.,-1.));
#114657=DIRECTION('ref_axis',(-1.,0.,1.4081690688991E-16));
#114658=DIRECTION('',(0.334565204279774,-0.371579218892547,0.866022521746656));
#114659=DIRECTION('center_axis',(-1.4081690688991E-16,0.,-1.));
#114660=DIRECTION('ref_axis',(-1.,0.,1.40816906889911E-16));
#114661=DIRECTION('',(-0.587785252292466,0.809016994374953,8.27701011433307E-17));
#114662=DIRECTION('center_axis',(1.4081690688991E-16,0.,1.));
#114663=DIRECTION('ref_axis',(-1.,2.48689957516035E-14,1.4081690688991E-16));
#114664=DIRECTION('',(0.669130606358852,-0.7431448254774,-9.42249022928238E-17));
#114665=DIRECTION('center_axis',(-1.4081690688991E-16,0.,-1.));
#114666=DIRECTION('ref_axis',(-1.,0.,1.17174841180864E-16));
#114667=DIRECTION('center_axis',(0.808387450334136,0.588650770899371,7.86457201793794E-6));
#114668=DIRECTION('ref_axis',(5.49541672851605E-6,5.81354221112889E-6,-0.999999999968002));
#114669=DIRECTION('center_axis',(-0.743860540860193,-0.668334867928743,
7.86457217253649E-6));
#114670=DIRECTION('ref_axis',(0.566774825493203,-0.630829867029694,-0.529924500330422));
#114671=DIRECTION('center_axis',(-1.4081690688991E-16,0.,-1.));
#114672=DIRECTION('ref_axis',(-1.,0.,1.13676889660403E-16));
#114673=DIRECTION('center_axis',(0.808414296622801,0.588613901399208,-9.7705831004133E-6));
#114674=DIRECTION('ref_axis',(0.514822445316052,-0.707075657763321,-0.484769908304308));
#114675=DIRECTION('center_axis',(-0.7438300586801,-0.668368793188683,-9.77051765796924E-6));
#114676=DIRECTION('ref_axis',(0.584591780668461,-0.650587230627073,-0.4847563360286));
#114677=DIRECTION('center_axis',(-1.4081690688991E-16,0.,-1.));
#114678=DIRECTION('ref_axis',(-1.,0.,1.15974593313694E-16));
#114679=DIRECTION('center_axis',(-0.810541512988718,-0.585681189207989,
1.81624798788288E-5));
#114680=DIRECTION('ref_axis',(0.506765009439008,-0.701311531423695,0.501349539842647));
#114681=DIRECTION('center_axis',(0.74140371840874,0.671059256698644,1.81316453410639E-5));
#114682=DIRECTION('ref_axis',(0.581789246428454,-0.642789354378472,0.498340364247086));
#114683=DIRECTION('center_axis',(-1.4081690688991E-16,0.,-1.));
#114684=DIRECTION('ref_axis',(-1.,0.,1.16261524579732E-16));
#114685=DIRECTION('center_axis',(-0.810549426620236,-0.585670237133129,
1.84940495645244E-5));
#114686=DIRECTION('ref_axis',(0.507758105720992,-0.702737191805956,-0.498339387694078));
#114687=DIRECTION('center_axis',(0.74139465132122,0.671069274105948,1.85257164118208E-5));
#114688=DIRECTION('ref_axis',(0.58064651661672,-0.641482109967248,-0.50134850686208));
#114689=DIRECTION('center_axis',(-1.4081690688991E-16,0.,-1.));
#114690=DIRECTION('ref_axis',(-1.,0.,1.40816906889911E-16));
#114691=DIRECTION('center_axis',(-1.4081690688991E-16,0.,-1.));
#114692=DIRECTION('ref_axis',(-1.,0.,1.4081690688991E-16));
#114693=DIRECTION('',(-0.669130606358852,0.7431448254774,9.42249022928238E-17));
#114694=DIRECTION('center_axis',(-1.4081690688991E-16,0.,-1.));
#114695=DIRECTION('ref_axis',(-1.,0.,1.4081690688991E-16));
#114696=DIRECTION('center_axis',(-1.4081690688991E-16,0.,-1.));
#114697=DIRECTION('ref_axis',(-1.,0.,1.4081690688991E-16));
#114698=DIRECTION('center_axis',(-1.4081690688991E-16,0.,-1.));
#114699=DIRECTION('ref_axis',(-1.,0.,1.4081690688991E-16));
#114700=DIRECTION('',(0.743144825477389,-0.669130606358864,-1.04647355694968E-16));
#114701=DIRECTION('center_axis',(1.4081690688991E-16,0.,1.));
#114702=DIRECTION('ref_axis',(1.,0.,-1.4081690688991E-16));
#114703=DIRECTION('',(-0.334565226058171,0.371579467697561,0.866022406579785));
#114704=DIRECTION('center_axis',(1.4081690688991E-16,0.,1.));
#114705=DIRECTION('ref_axis',(-1.,7.105427357601E-15,1.40816906889911E-16));
#114706=DIRECTION('',(0.371579467697514,-0.334565226058178,-0.866022406579802));
#114707=DIRECTION('center_axis',(-1.4081690688991E-16,0.,-1.));
#114708=DIRECTION('ref_axis',(-1.,0.,1.40816906889911E-16));
#114709=DIRECTION('center_axis',(-1.4081690688991E-16,0.,-1.));
#114710=DIRECTION('ref_axis',(-1.,0.,1.4081690688991E-16));
#114711=DIRECTION('',(-0.669130606358852,0.7431448254774,9.42249022928238E-17));
#114712=DIRECTION('center_axis',(1.4081690688991E-16,0.,1.));
#114713=DIRECTION('ref_axis',(-1.,-3.90798504668055E-14,1.4081690688991E-16));
#114714=DIRECTION('',(0.743144825477389,-0.669130606358864,-1.04647355694968E-16));
#114715=DIRECTION('center_axis',(-1.4081690688991E-16,0.,-1.));
#114716=DIRECTION('ref_axis',(-1.,0.,1.4081690688991E-16));
#114717=DIRECTION('center_axis',(-1.4081690688991E-16,0.,-1.));
#114718=DIRECTION('ref_axis',(1.,0.,-1.4081690688991E-16));
#114719=DIRECTION('',(-0.3345720823863,0.371573025817577,-0.866022521746672));
#114720=DIRECTION('center_axis',(-1.4081690688991E-16,0.,-1.));
#114721=DIRECTION('ref_axis',(-1.,0.,1.4081690688991E-16));
#114722=DIRECTION('center_axis',(-1.4081690688991E-16,0.,-1.));
#114723=DIRECTION('ref_axis',(-1.,0.,1.4081690688991E-16));
#114724=DIRECTION('center_axis',(-1.4081690688991E-16,0.,-1.));
#114725=DIRECTION('ref_axis',(-1.,0.,1.4081690688991E-16));
#114726=DIRECTION('',(0.371573025817621,-0.334572082386318,0.866022521746647));
#114727=DIRECTION('center_axis',(-1.4081690688991E-16,0.,-1.));
#114728=DIRECTION('ref_axis',(-1.,0.,1.40816906889911E-16));
#114729=DIRECTION('',(-0.669130606358852,0.7431448254774,9.42249022928238E-17));
#114730=DIRECTION('center_axis',(1.4081690688991E-16,0.,1.));
#114731=DIRECTION('ref_axis',(-1.,-3.19744231092045E-14,1.4081690688991E-16));
#114732=DIRECTION('',(0.743144825477389,-0.669130606358864,-1.04647355694968E-16));
#114733=DIRECTION('center_axis',(-1.4081690688991E-16,0.,-1.));
#114734=DIRECTION('ref_axis',(-1.,0.,1.17174841180864E-16));
#114735=DIRECTION('center_axis',(0.742428258814843,0.669925578293073,7.86457196552063E-6));
#114736=DIRECTION('ref_axis',(4.85763160251991E-6,6.35612243375601E-6,-0.999999999968002));
#114737=DIRECTION('center_axis',(-0.669925578293223,-0.742428258814708,
7.86457226896801E-6));
#114738=DIRECTION('ref_axis',(0.62960965028037,-0.568130013485746,-0.529924500330487));
#114739=DIRECTION('center_axis',(-1.4081690688991E-16,0.,-1.));
#114740=DIRECTION('ref_axis',(-1.,0.,1.13676889660403E-16));
#114741=DIRECTION('center_axis',(0.742458811945264,0.669891716973245,-9.77059280552686E-6));
#114742=DIRECTION('ref_axis',(0.585911726013662,-0.649388624262771,-0.484769908304752));
#114743=DIRECTION('center_axis',(-0.66989171694181,-0.742458811973628,-9.77051631735247E-6));
#114744=DIRECTION('ref_axis',(0.649394209166982,-0.585916765234243,-0.484756336026494));
#114745=DIRECTION('center_axis',(-1.4081690688991E-16,0.,-1.));
#114746=DIRECTION('ref_axis',(-1.,0.,1.15974593313694E-16));
#114747=DIRECTION('center_axis',(-0.744880927099423,-0.667197425140137,
1.81624796016105E-5));
#114748=DIRECTION('ref_axis',(0.577295914344574,-0.644498305799945,0.501349539844272));
#114749=DIRECTION('center_axis',(0.667197438400719,0.744880915222536,1.81316452123543E-5));
#114750=DIRECTION('ref_axis',(0.645791927479624,-0.578454551163014,0.498340364250127));
#114751=DIRECTION('center_axis',(-1.4081690688991E-16,0.,-1.));
#114752=DIRECTION('ref_axis',(-1.,0.,1.16261524579732E-16));
#114753=DIRECTION('center_axis',(-0.744889942181918,-0.667187360262609,
1.84940520599162E-5));
#114754=DIRECTION('ref_axis',(0.578432592428309,-0.645812349435162,-0.498339387700493));
#114755=DIRECTION('center_axis',(0.667187373880019,0.74488992998421,1.85257177449103E-5));
#114756=DIRECTION('ref_axis',(0.644518813413743,-0.577273915766274,-0.50134850686086));
#114757=DIRECTION('center_axis',(-1.4081690688991E-16,0.,-1.));
#114758=DIRECTION('ref_axis',(-1.,0.,1.40816906889911E-16));
#114759=DIRECTION('center_axis',(-1.4081690688991E-16,0.,-1.));
#114760=DIRECTION('ref_axis',(-1.,0.,1.4081690688991E-16));
#114761=DIRECTION('',(-0.743144825477389,0.669130606358864,1.04647355694968E-16));
#114762=DIRECTION('center_axis',(-1.4081690688991E-16,0.,-1.));
#114763=DIRECTION('ref_axis',(-1.,0.,1.4081690688991E-16));
#114764=DIRECTION('center_axis',(-1.4081690688991E-16,0.,-1.));
#114765=DIRECTION('ref_axis',(-1.,0.,1.4081690688991E-16));
#114766=DIRECTION('center_axis',(-1.4081690688991E-16,0.,-1.));
#114767=DIRECTION('ref_axis',(-1.,0.,1.4081690688991E-16));
#114768=DIRECTION('',(0.809016994374943,-0.58778525229248,-1.13923270769252E-16));
#114769=DIRECTION('center_axis',(1.4081690688991E-16,0.,1.));
#114770=DIRECTION('ref_axis',(1.,0.,-1.4081690688991E-16));
#114771=DIRECTION('',(-0.371573073483894,0.334572327551861,0.866022406579797));
#114772=DIRECTION('center_axis',(1.4081690688991E-16,0.,1.));
#114773=DIRECTION('ref_axis',(-1.,2.66453525910038E-14,1.40816906889911E-16));
#114774=DIRECTION('',(0.404515505437159,-0.293891812003487,-0.866022406579776));
#114775=DIRECTION('center_axis',(-1.4081690688991E-16,0.,-1.));
#114776=DIRECTION('ref_axis',(-1.,0.,1.40816906889911E-16));
#114777=DIRECTION('center_axis',(-1.4081690688991E-16,0.,-1.));
#114778=DIRECTION('ref_axis',(-1.,0.,1.4081690688991E-16));
#114779=DIRECTION('',(-0.743144825477389,0.669130606358864,1.04647355694968E-16));
#114780=DIRECTION('center_axis',(1.4081690688991E-16,0.,1.));
#114781=DIRECTION('ref_axis',(-1.,1.33226762955019E-14,1.4081690688991E-16));
#114782=DIRECTION('',(0.809016994374943,-0.58778525229248,-1.13923270769252E-16));
#114783=DIRECTION('center_axis',(-1.4081690688991E-16,0.,-1.));
#114784=DIRECTION('ref_axis',(-1.,0.,1.4081690688991E-16));
#114785=DIRECTION('center_axis',(-1.4081690688991E-16,0.,-1.));
#114786=DIRECTION('ref_axis',(1.,0.,-1.4081690688991E-16));
#114787=DIRECTION('',(-0.371579218892551,0.33456520427975,-0.866022521746664));
#114788=DIRECTION('center_axis',(-1.4081690688991E-16,0.,-1.));
#114789=DIRECTION('ref_axis',(-1.,0.,1.4081690688991E-16));
#114790=DIRECTION('center_axis',(-1.4081690688991E-16,0.,-1.));
#114791=DIRECTION('ref_axis',(-1.,0.,1.4081690688991E-16));
#114792=DIRECTION('center_axis',(-1.4081690688991E-16,0.,-1.));
#114793=DIRECTION('ref_axis',(-1.,0.,1.4081690688991E-16));
#114794=DIRECTION('',(0.404509815527948,-0.293899304131707,0.86602252174666));
#114795=DIRECTION('center_axis',(-1.4081690688991E-16,0.,-1.));
#114796=DIRECTION('ref_axis',(-1.,0.,1.40816906889911E-16));
#114797=DIRECTION('',(-0.743144825477389,0.669130606358864,1.04647355694968E-16));
#114798=DIRECTION('center_axis',(1.4081690688991E-16,0.,1.));
#114799=DIRECTION('ref_axis',(-1.,2.57571741713036E-14,1.4081690688991E-16));
#114800=DIRECTION('',(0.809016994374943,-0.58778525229248,-1.13923270769252E-16));
#114801=DIRECTION('center_axis',(-1.4081690688991E-16,0.,-1.));
#114802=DIRECTION('ref_axis',(-1.,0.,1.17174841180864E-16));
#114803=DIRECTION('center_axis',(0.668334867928844,0.743860540860102,7.86457191841109E-6));
#114804=DIRECTION('ref_axis',(4.16662522946725E-6,6.8290636700625E-6,-0.999999999968001));
#114805=DIRECTION('center_axis',(-0.588650770899511,-0.808387450334034,
7.86457230678758E-6));
#114806=DIRECTION('ref_axis',(0.685546339984867,-0.499205608625207,-0.529924500330462));
#114807=DIRECTION('center_axis',(-1.4081690688991E-16,0.,-1.));
#114808=DIRECTION('ref_axis',(-1.,0.,1.13676889660403E-16));
#114809=DIRECTION('center_axis',(0.668368793161135,0.743830058704852,-9.77058447225306E-6));
#114810=DIRECTION('ref_axis',(0.650581635232363,-0.584586753102607,-0.484769908302213));
#114811=DIRECTION('center_axis',(-0.588613901370769,-0.808414296643509,
-9.77051950914831E-6));
#114812=DIRECTION('ref_axis',(0.707081738814109,-0.514826873149292,-0.484756336027636));
#114813=DIRECTION('center_axis',(-1.4081690688991E-16,0.,-1.));
#114814=DIRECTION('ref_axis',(-1.,0.,1.15974593313694E-16));
#114815=DIRECTION('center_axis',(-0.671059269896554,-0.741403706462295,
1.8162479710228E-5));
#114816=DIRECTION('ref_axis',(0.641501844406933,-0.580623821869249,0.501349539842663));
#114817=DIRECTION('center_axis',(0.585681203637554,0.810541502562891,1.81316450912546E-5));
#114818=DIRECTION('ref_axis',(0.702719177034773,-0.5077820788376,0.498340364248107));
#114819=DIRECTION('center_axis',(-1.4081690688991E-16,0.,-1.));
#114820=DIRECTION('ref_axis',(-1.,0.,1.16261524579732E-16));
#114821=DIRECTION('center_axis',(-0.671069287650237,-0.741394639062472,
1.84940740096905E-5));
#114822=DIRECTION('ref_axis',(0.642769650611826,-0.581811851823278,-0.498339387697099));
#114823=DIRECTION('center_axis',(0.585670251949479,0.810549415913818,1.8525712039311E-5));
#114824=DIRECTION('ref_axis',(0.701329627217096,-0.506740987741917,-0.501348506859126));
#114825=DIRECTION('center_axis',(-1.4081690688991E-16,0.,-1.));
#114826=DIRECTION('ref_axis',(-1.,0.,1.40816906889911E-16));
#114827=DIRECTION('center_axis',(-1.4081690688991E-16,0.,-1.));
#114828=DIRECTION('ref_axis',(-1.,0.,1.4081690688991E-16));
#114829=DIRECTION('',(-0.809016994374943,0.58778525229248,1.13923270769252E-16));
#114830=DIRECTION('center_axis',(-1.4081690688991E-16,0.,-1.));
#114831=DIRECTION('ref_axis',(-1.,0.,1.4081690688991E-16));
#114832=DIRECTION('center_axis',(-1.4081690688991E-16,0.,-1.));
#114833=DIRECTION('ref_axis',(-1.,0.,1.4081690688991E-16));
#114834=DIRECTION('center_axis',(-1.4081690688991E-16,0.,-1.));
#114835=DIRECTION('ref_axis',(-1.,0.,1.4081690688991E-16));
#114836=DIRECTION('',(0.866025403784435,-0.500000000000007,-1.2195101864901E-16));
#114837=DIRECTION('center_axis',(1.4081690688991E-16,0.,1.));
#114838=DIRECTION('ref_axis',(1.,0.,-1.4081690688991E-16));
#114839=DIRECTION('',(-0.404509888559932,0.29389954297172,0.866022406579787));
#114840=DIRECTION('center_axis',(1.4081690688991E-16,0.,1.));
#114841=DIRECTION('ref_axis',(-1.,7.105427357601E-15,1.40816906889911E-16));
#114842=DIRECTION('',(0.433019586648901,-0.249998457755605,-0.86602240657978));
#114843=DIRECTION('center_axis',(-1.4081690688991E-16,0.,-1.));
#114844=DIRECTION('ref_axis',(-1.,0.,1.40816906889911E-16));
#114845=DIRECTION('center_axis',(-1.4081690688991E-16,0.,-1.));
#114846=DIRECTION('ref_axis',(-1.,0.,1.4081690688991E-16));
#114847=DIRECTION('',(-0.809016994374943,0.58778525229248,1.13923270769252E-16));
#114848=DIRECTION('center_axis',(1.4081690688991E-16,0.,1.));
#114849=DIRECTION('ref_axis',(-1.,-3.99680288865056E-14,1.4081690688991E-16));
#114850=DIRECTION('',(0.866025403784435,-0.500000000000007,-1.2195101864901E-16));
#114851=DIRECTION('center_axis',(-1.4081690688991E-16,0.,-1.));
#114852=DIRECTION('ref_axis',(-1.,0.,1.4081690688991E-16));
#114853=DIRECTION('center_axis',(-1.4081690688991E-16,0.,-1.));
#114854=DIRECTION('ref_axis',(1.,0.,-1.4081690688991E-16));
#114855=DIRECTION('',(-0.404515255718706,0.293891816351498,-0.866022521746661));
#114856=DIRECTION('center_axis',(-1.4081690688991E-16,0.,-1.));
#114857=DIRECTION('ref_axis',(-1.,0.,1.4081690688991E-16));
#114858=DIRECTION('center_axis',(-1.4081690688991E-16,0.,-1.));
#114859=DIRECTION('ref_axis',(-1.,0.,1.4081690688991E-16));
#114860=DIRECTION('center_axis',(-1.4081690688991E-16,0.,-1.));
#114861=DIRECTION('ref_axis',(-1.,0.,1.4081690688991E-16));
#114862=DIRECTION('',(0.433014711050233,-0.250006503598672,0.866022521746663));
#114863=DIRECTION('center_axis',(-1.4081690688991E-16,0.,-1.));
#114864=DIRECTION('ref_axis',(-1.,0.,1.40816906889911E-16));
#114865=DIRECTION('',(-0.809016994374943,0.58778525229248,1.13923270769252E-16));
#114866=DIRECTION('center_axis',(1.4081690688991E-16,0.,1.));
#114867=DIRECTION('ref_axis',(-1.,-2.66453525910038E-14,1.4081690688991E-16));
#114868=DIRECTION('',(0.866025403784435,-0.500000000000007,-1.2195101864901E-16));
#114869=DIRECTION('center_axis',(-1.4081690688991E-16,0.,-1.));
#114870=DIRECTION('ref_axis',(-1.,0.,1.17174841180864E-16));
#114871=DIRECTION('center_axis',(0.586919060371726,0.809645611678665,7.86457193544097E-6));
#114872=DIRECTION('ref_axis',(3.42996849075291E-6,7.2271843029038E-6,-0.999999999968002));
#114873=DIRECTION('center_axis',(-0.50092658247667,-0.865489779781594,7.86457223048433E-6));
#114874=DIRECTION('ref_axis',(0.733972040528744,-0.424811802650955,-0.529924500330489));
#114875=DIRECTION('center_axis',(-1.4081690688991E-16,0.,-1.));
#114876=DIRECTION('ref_axis',(-1.,0.,1.13676889660403E-16));
#114877=DIRECTION('center_axis',(0.586955986005752,0.809618842663973,-9.77059599688668E-6));
#114878=DIRECTION('ref_axis',(0.708123635911378,-0.513380027141705,-0.484769908302518));
#114879=DIRECTION('center_axis',(-0.500887108715761,-0.865512625111213,
-9.77051146875296E-6));
#114880=DIRECTION('ref_axis',(0.757022332964799,-0.438096430108037,-0.484756336027831));
#114881=DIRECTION('center_axis',(-1.4081690688991E-16,0.,-1.));
#114882=DIRECTION('ref_axis',(-1.,0.,1.15974593313694E-16));
#114883=DIRECTION('center_axis',(-0.589885346904536,-0.807487013627736,
1.81624796204011E-5));
#114884=DIRECTION('ref_axis',(0.69867934601963,-0.510387901843116,0.501349539839984));
#114885=DIRECTION('center_axis',(0.497748123045631,0.867321627584482,1.8131645060743E-5));
#114886=DIRECTION('ref_axis',(0.751947288228587,-0.43154623979347,0.498340364254986));
#114887=DIRECTION('center_axis',(-1.4081690688991E-16,0.,-1.));
#114888=DIRECTION('ref_axis',(-1.,0.,1.16261524579732E-16));
#114889=DIRECTION('center_axis',(-0.589896257585103,-0.807479043037687,
1.8494065967643E-5));
#114890=DIRECTION('ref_axis',(0.700064389990716,-0.511436901807441,-0.498339387703332));
#114891=DIRECTION('center_axis',(0.497736404185315,0.86732835282001,1.85257193500676E-5));
#114892=DIRECTION('ref_axis',(0.750456526859374,-0.430656099411711,-0.501348506862897));
#114893=DIRECTION('center_axis',(-1.4081690688991E-16,0.,-1.));
#114894=DIRECTION('ref_axis',(-1.,0.,1.40816906889911E-16));
#114895=DIRECTION('center_axis',(-1.4081690688991E-16,0.,-1.));
#114896=DIRECTION('ref_axis',(-1.,0.,1.4081690688991E-16));
#114897=DIRECTION('',(-0.866025403784435,0.500000000000007,1.2195101864901E-16));
#114898=DIRECTION('center_axis',(-1.4081690688991E-16,0.,-1.));
#114899=DIRECTION('ref_axis',(-1.,0.,1.4081690688991E-16));
#114900=DIRECTION('center_axis',(-1.4081690688991E-16,0.,-1.));
#114901=DIRECTION('ref_axis',(-1.,0.,1.4081690688991E-16));
#114902=DIRECTION('center_axis',(-1.4081690688991E-16,0.,-1.));
#114903=DIRECTION('ref_axis',(-1.,0.,1.4081690688991E-16));
#114904=DIRECTION('',(0.913545457642598,-0.406736643075807,-1.28642645648558E-16));
#114905=DIRECTION('center_axis',(1.4081690688991E-16,0.,1.));
#114906=DIRECTION('ref_axis',(1.,0.,-1.4081690688991E-16));
#114907=DIRECTION('',(-0.433014808647733,0.250006733496379,0.866022406579782));
#114908=DIRECTION('center_axis',(1.4081690688991E-16,0.,1.));
#114909=DIRECTION('ref_axis',(-1.,-7.105427357601E-15,1.40816906889911E-16));
#114910=DIRECTION('',(0.456779414654109,-0.203366068089036,-0.866022406579792));
#114911=DIRECTION('center_axis',(-1.4081690688991E-16,0.,-1.));
#114912=DIRECTION('ref_axis',(-1.,0.,1.40816906889911E-16));
#114913=DIRECTION('center_axis',(-1.4081690688991E-16,0.,-1.));
#114914=DIRECTION('ref_axis',(-1.,0.,1.4081690688991E-16));
#114915=DIRECTION('',(-0.866025403784435,0.500000000000007,1.2195101864901E-16));
#114916=DIRECTION('center_axis',(1.4081690688991E-16,0.,1.));
#114917=DIRECTION('ref_axis',(-1.,-7.105427357601E-15,1.4081690688991E-16));
#114918=DIRECTION('',(0.913545457642598,-0.406736643075807,-1.28642645648558E-16));
#114919=DIRECTION('center_axis',(-1.4081690688991E-16,0.,-1.));
#114920=DIRECTION('ref_axis',(-1.,0.,1.4081690688991E-16));
#114921=DIRECTION('center_axis',(-1.4081690688991E-16,0.,-1.));
#114922=DIRECTION('ref_axis',(1.,0.,-1.4081690688991E-16));
#114923=DIRECTION('',(-0.433019338752863,0.249998488182549,-0.866022521746677));
#114924=DIRECTION('center_axis',(-1.4081690688991E-16,0.,-1.));
#114925=DIRECTION('ref_axis',(-1.,0.,1.4081690688991E-16));
#114926=DIRECTION('center_axis',(-1.4081690688991E-16,0.,-1.));
#114927=DIRECTION('ref_axis',(-1.,0.,1.4081690688991E-16));
#114928=DIRECTION('center_axis',(-1.4081690688991E-16,0.,-1.));
#114929=DIRECTION('ref_axis',(-1.,0.,1.4081690688991E-16));
#114930=DIRECTION('',(0.456775406784116,-0.203374579494969,0.866022521746663));
#114931=DIRECTION('center_axis',(-1.4081690688991E-16,0.,-1.));
#114932=DIRECTION('ref_axis',(-1.,0.,1.40816906889911E-16));
#114933=DIRECTION('',(-0.866025403784435,0.500000000000007,1.2195101864901E-16));
#114934=DIRECTION('center_axis',(1.4081690688991E-16,0.,1.));
#114935=DIRECTION('ref_axis',(-1.,0.,1.4081690688991E-16));
#114936=DIRECTION('',(0.913545457642598,-0.406736643075807,-1.28642645648558E-16));
#114937=DIRECTION('center_axis',(-1.4081690688991E-16,0.,-1.));
#114938=DIRECTION('ref_axis',(-1.,0.,1.17174841180864E-16));
#114939=DIRECTION('center_axis',(0.499072844768408,0.866560035746466,7.86457209402E-6));
#114940=DIRECTION('ref_axis',(2.65573233462647E-6,7.54612252265976E-6,-0.999999999968002));
#114941=DIRECTION('center_axis',(-0.407714137590654,-0.913109622086449,
7.86457233598189E-6));
#114942=DIRECTION('ref_axis',(0.774356189803017,-0.345763669669441,-0.529924500330448));
#114943=DIRECTION('center_axis',(-1.4081690688991E-16,0.,-1.));
#114944=DIRECTION('ref_axis',(-1.,0.,1.13676889660403E-16));
#114945=DIRECTION('center_axis',(0.499112366250355,0.866537273151309,-9.77058284535403E-6));
#114946=DIRECTION('ref_axis',(0.757907285851051,-0.436548602171899,-0.484769908302541));
#114947=DIRECTION('center_axis',(-0.40767249208604,-0.913128216134457,-9.77051569036097E-6));
#114948=DIRECTION('ref_axis',(0.798668832019631,-0.356566110901516,-0.484756336025602));
#114949=DIRECTION('center_axis',(-1.4081690688991E-16,0.,-1.));
#114950=DIRECTION('ref_axis',(-1.,0.,1.15974593313694E-16));
#114951=DIRECTION('center_axis',(-0.5022485166105,-0.864723324094289,1.81624798677622E-5));
#114952=DIRECTION('ref_axis',(0.748201970507648,-0.434560065157467,0.501349539841027));
#114953=DIRECTION('center_axis',(0.404361609857045,0.914599195355573,1.81316452956218E-5));
#114954=DIRECTION('ref_axis',(0.79293690758283,-0.350582289842627,0.498340364250858));
#114955=DIRECTION('center_axis',(-1.4081690688991E-16,0.,-1.));
#114956=DIRECTION('ref_axis',(-1.,0.,1.16261524579732E-16));
#114957=DIRECTION('center_axis',(-0.502260200672834,-0.86471653764575,1.84940694697466E-5));
#114958=DIRECTION('ref_axis',(0.749689077418704,-0.435458542073202,-0.498339387701367));
#114959=DIRECTION('center_axis',(0.404349252216125,0.914604658794748,1.85257207050329E-5));
#114960=DIRECTION('ref_axis',(0.791361267750536,-0.349852852736373,-0.50134850686572));
#114961=DIRECTION('center_axis',(-1.4081690688991E-16,0.,-1.));
#114962=DIRECTION('ref_axis',(-1.,0.,1.40816906889911E-16));
#114963=DIRECTION('center_axis',(-1.4081690688991E-16,0.,-1.));
#114964=DIRECTION('ref_axis',(-1.,0.,1.4081690688991E-16));
#114965=DIRECTION('',(-0.913545457642598,0.406736643075807,1.28642645648558E-16));
#114966=DIRECTION('center_axis',(-1.4081690688991E-16,0.,-1.));
#114967=DIRECTION('ref_axis',(-1.,0.,1.4081690688991E-16));
#114968=DIRECTION('center_axis',(-1.4081690688991E-16,0.,-1.));
#114969=DIRECTION('ref_axis',(-1.,0.,1.4081690688991E-16));
#114970=DIRECTION('center_axis',(-1.4081690688991E-16,0.,-1.));
#114971=DIRECTION('ref_axis',(-1.,0.,1.4081690688991E-16));
#114972=DIRECTION('',(0.951056516295151,-0.309016994374955,-1.33924836902177E-16));
#114973=DIRECTION('center_axis',(1.4081690688991E-16,0.,1.));
#114974=DIRECTION('ref_axis',(1.,0.,-1.4081690688991E-16));
#114975=DIRECTION('',(-0.45677552787782,0.203374797931578,0.866022406579777));
#114976=DIRECTION('center_axis',(1.4081690688991E-16,0.,1.));
#114977=DIRECTION('ref_axis',(-1.,2.1316282072803E-14,1.40816906889911E-16));
#114978=DIRECTION('',(0.475534671805163,-0.154505557223394,-0.866022406579786));
#114979=DIRECTION('center_axis',(-1.4081690688991E-16,0.,-1.));
#114980=DIRECTION('ref_axis',(-1.,0.,1.40816906889911E-16));
#114981=DIRECTION('center_axis',(-1.4081690688991E-16,0.,-1.));
#114982=DIRECTION('ref_axis',(-1.,0.,1.4081690688991E-16));
#114983=DIRECTION('',(-0.913545457642598,0.406736643075807,1.28642645648558E-16));
#114984=DIRECTION('center_axis',(1.4081690688991E-16,0.,1.));
#114985=DIRECTION('ref_axis',(-1.,1.77635683940025E-14,1.4081690688991E-16));
#114986=DIRECTION('',(0.951056516295151,-0.309016994374955,-1.33924836902177E-16));
#114987=DIRECTION('center_axis',(-1.4081690688991E-16,0.,-1.));
#114988=DIRECTION('ref_axis',(-1.,0.,1.4081690688991E-16));
#114989=DIRECTION('center_axis',(-1.4081690688991E-16,0.,-1.));
#114990=DIRECTION('ref_axis',(1.,0.,-1.4081690688991E-16));
#114991=DIRECTION('',(-0.456779171296622,0.203366124261496,-0.866022521746652));
#114992=DIRECTION('center_axis',(-1.4081690688991E-16,0.,-1.));
#114993=DIRECTION('ref_axis',(-1.,0.,1.4081690688991E-16));
#114994=DIRECTION('center_axis',(-1.4081690688991E-16,0.,-1.));
#114995=DIRECTION('ref_axis',(-1.,0.,1.4081690688991E-16));
#114996=DIRECTION('center_axis',(-1.4081690688991E-16,0.,-1.));
#114997=DIRECTION('ref_axis',(-1.,0.,1.4081690688991E-16));
#114998=DIRECTION('',(0.475531575574881,-0.154514440939472,0.866022521746654));
#114999=DIRECTION('center_axis',(-1.4081690688991E-16,0.,-1.));
#115000=DIRECTION('ref_axis',(-1.,0.,1.40816906889911E-16));
#115001=DIRECTION('',(-0.913545457642598,0.406736643075807,1.28642645648558E-16));
#115002=DIRECTION('center_axis',(1.4081690688991E-16,0.,1.));
#115003=DIRECTION('ref_axis',(-1.,2.04281036531029E-14,1.4081690688991E-16));
#115004=DIRECTION('',(0.951056516295151,-0.309016994374955,-1.33924836902177E-16));
#115005=DIRECTION('center_axis',(-1.4081690688991E-16,0.,-1.));
#115006=DIRECTION('ref_axis',(-1.,0.,1.17174841180864E-16));
#115007=DIRECTION('center_axis',(0.405758682640175,0.913980246723231,7.86457213173083E-6));
#115008=DIRECTION('ref_axis',(1.85239945587365E-6,7.78238369388909E-6,-0.999999999968002));
#115009=DIRECTION('center_axis',(-0.310034691293475,-0.950725244291277,
7.86457228997841E-6));
#115010=DIRECTION('ref_axis',(0.806256330617388,-0.262927277567195,-0.529924500330461));
#115011=DIRECTION('center_axis',(-1.4081690688991E-16,0.,-1.));
#115012=DIRECTION('ref_axis',(-1.,0.,1.13676889660403E-16));
#115013=DIRECTION('center_axis',(0.405800366956845,0.913961739944417,-9.7705859397404E-6));
#115014=DIRECTION('ref_axis',(0.799387144965416,-0.354934259363339,-0.484769908301082));
#115015=DIRECTION('center_axis',(-0.30999133032007,-0.950739383338531,-9.77051572543388E-6));
#115016=DIRECTION('ref_axis',(0.831564948215717,-0.27112917876648,-0.48475633602915));
#115017=DIRECTION('center_axis',(-1.4081690688991E-16,0.,-1.));
#115018=DIRECTION('ref_axis',(-1.,0.,1.15974593313694E-16));
#115019=DIRECTION('center_axis',(-0.409108946466016,-0.9124855448672,1.81624797290291E-5));
#115020=DIRECTION('ref_axis',(0.789527137637376,-0.353971097461394,0.501349539838333));
#115021=DIRECTION('center_axis',(0.306544826252831,0.951856222950118,1.81316453078655E-5));
#115022=DIRECTION('ref_axis',(0.825238944245296,-0.265777286959786,0.49834036424637));
#115023=DIRECTION('center_axis',(-1.4081690688991E-16,0.,-1.));
#115024=DIRECTION('ref_axis',(-1.,0.,1.16261524579732E-16));
#115025=DIRECTION('center_axis',(-0.409121275899226,-0.912480016912458,
1.84940689712829E-5));
#115026=DIRECTION('ref_axis',(0.791100014430625,-0.354709207425649,-0.49833938770213));
#115027=DIRECTION('center_axis',(0.306531965219087,0.951860364736195,1.85257126434399E-5));
#115028=DIRECTION('ref_axis',(0.823595688995553,-0.265216544997509,-0.501348506856782));
#115029=DIRECTION('center_axis',(-1.4081690688991E-16,0.,-1.));
#115030=DIRECTION('ref_axis',(-1.,0.,1.40816906889911E-16));
#115031=DIRECTION('center_axis',(-1.4081690688991E-16,0.,-1.));
#115032=DIRECTION('ref_axis',(-1.,0.,1.4081690688991E-16));
#115033=DIRECTION('',(-0.951056516295151,0.309016994374955,1.33924836902177E-16));
#115034=DIRECTION('center_axis',(-1.4081690688991E-16,0.,-1.));
#115035=DIRECTION('ref_axis',(-1.,0.,1.4081690688991E-16));
#115036=DIRECTION('center_axis',(-1.4081690688991E-16,0.,-1.));
#115037=DIRECTION('ref_axis',(-1.,0.,1.4081690688991E-16));
#115038=DIRECTION('center_axis',(-1.4081690688991E-16,0.,-1.));
#115039=DIRECTION('ref_axis',(-1.,0.,1.4081690688991E-16));
#115040=DIRECTION('',(0.978147600733804,-0.207911690817766,-1.37739719617121E-16));
#115041=DIRECTION('center_axis',(1.4081690688991E-16,0.,1.));
#115042=DIRECTION('ref_axis',(1.,0.,-1.4081690688991E-16));
#115043=DIRECTION('',(-0.475531718838045,0.154514645521707,0.866022406579781));
#115044=DIRECTION('center_axis',(1.4081690688991E-16,0.,1.));
#115045=DIRECTION('ref_axis',(-1.,-4.08562073062058E-14,1.40816906889911E-16));
#115046=DIRECTION('',(0.489079871579872,-0.103952251140486,-0.866022406579784));
#115047=DIRECTION('center_axis',(-1.4081690688991E-16,0.,-1.));
#115048=DIRECTION('ref_axis',(-1.,0.,1.40816906889911E-16));
#115049=DIRECTION('center_axis',(-1.4081690688991E-16,0.,-1.));
#115050=DIRECTION('ref_axis',(-1.,0.,1.4081690688991E-16));
#115051=DIRECTION('',(-0.951056516295151,0.309016994374955,1.33924836902177E-16));
#115052=DIRECTION('center_axis',(1.4081690688991E-16,0.,1.));
#115053=DIRECTION('ref_axis',(-1.,-3.28626015289046E-14,1.4081690688991E-16));
#115054=DIRECTION('',(0.978147600733804,-0.207911690817766,-1.37739719617121E-16));
#115055=DIRECTION('center_axis',(-1.4081690688991E-16,0.,-1.));
#115056=DIRECTION('ref_axis',(-1.,0.,1.4081690688991E-16));
#115057=DIRECTION('center_axis',(-1.4081690688991E-16,0.,-1.));
#115058=DIRECTION('ref_axis',(1.,0.,-1.4081690688991E-16));
#115059=DIRECTION('',(-0.475534435652379,0.154505638525967,-0.866022521746667));
#115060=DIRECTION('center_axis',(-1.4081690688991E-16,0.,-1.));
#115061=DIRECTION('ref_axis',(-1.,0.,1.4081690688991E-16));
#115062=DIRECTION('center_axis',(-1.4081690688991E-16,0.,-1.));
#115063=DIRECTION('ref_axis',(-1.,0.,1.4081690688991E-16));
#115064=DIRECTION('center_axis',(-1.4081690688991E-16,0.,-1.));
#115065=DIRECTION('ref_axis',(-1.,0.,1.4081690688991E-16));
#115066=DIRECTION('',(0.489077720912262,-0.103961409834809,0.86602252174665));
#115067=DIRECTION('center_axis',(-1.4081690688991E-16,0.,-1.));
#115068=DIRECTION('ref_axis',(-1.,0.,1.40816906889911E-16));
#115069=DIRECTION('',(-0.951056516295151,0.309016994374955,1.33924836902177E-16));
#115070=DIRECTION('center_axis',(1.4081690688991E-16,0.,1.));
#115071=DIRECTION('ref_axis',(-1.,-2.66453525910038E-14,1.4081690688991E-16));
#115072=DIRECTION('',(0.978147600733804,-0.207911690817766,-1.37739719617121E-16));
#115073=DIRECTION('center_axis',(-1.4081690688991E-16,0.,-1.));
#115074=DIRECTION('ref_axis',(-1.,0.,1.17174841180864E-16));
#115075=DIRECTION('center_axis',(0.307998943474507,0.951386698854223,7.86457204724389E-6));
#115076=DIRECTION('ref_axis',(1.02877119897224E-6,7.93337936481566E-6,-0.999999999968002));
#115077=DIRECTION('center_axis',(-0.208958440039582,-0.977924521767592,
7.8645723171832E-6));
#115078=DIRECTION('ref_axis',(0.829322958353485,-0.177210199190913,-0.529924500330509));
#115079=DIRECTION('center_axis',(-1.4081690688991E-16,0.,-1.));
#115080=DIRECTION('ref_axis',(-1.,0.,1.13676889660403E-16));
#115081=DIRECTION('center_axis',(0.308042333922939,0.951372650655801,-9.77059018674394E-6));
#115082=DIRECTION('ref_axis',(0.832108751234766,-0.269431182533443,-0.484769908304082));
#115083=DIRECTION('center_axis',(-0.208913838669525,-0.97793405090369,-9.77051623324827E-6));
#115084=DIRECTION('ref_axis',(0.855350264824845,-0.182721698612272,-0.484756336029055));
#115085=DIRECTION('center_axis',(-1.4081690688991E-16,0.,-1.));
#115086=DIRECTION('ref_axis',(-1.,0.,1.15974593313694E-16));
#115087=DIRECTION('center_axis',(-0.311487093092559,-0.950250383060629,
1.81624797254184E-5));
#115088=DIRECTION('ref_axis',(0.822202080228268,-0.26950394834807,0.501349539835342));
#115089=DIRECTION('center_axis',(0.205369473383598,0.978684514577291,1.81316452366172E-5));
#115090=DIRECTION('ref_axis',(0.848499490337296,-0.178060372501941,0.498340364251));
#115091=DIRECTION('center_axis',(-1.4081690688991E-16,0.,-1.));
#115092=DIRECTION('ref_axis',(-1.,0.,1.16261524579732E-16));
#115093=DIRECTION('center_axis',(-0.311499932817119,-0.95024617416378,1.84940604347653E-5));
#115094=DIRECTION('ref_axis',(0.82384349413835,-0.270073604474662,-0.498339387698762));
#115095=DIRECTION('center_axis',(0.205356249868039,0.978687289330424,1.85257103484312E-5));
#115096=DIRECTION('ref_axis',(0.846806623518866,-0.177674469289364,-0.501348506856578));
#115097=DIRECTION('center_axis',(-1.4081690688991E-16,0.,-1.));
#115098=DIRECTION('ref_axis',(-1.,0.,1.40816906889911E-16));
#115099=DIRECTION('center_axis',(-1.4081690688991E-16,0.,-1.));
#115100=DIRECTION('ref_axis',(-1.,0.,1.4081690688991E-16));
#115101=DIRECTION('',(-0.978147600733804,0.207911690817766,1.37739719617121E-16));
#115102=DIRECTION('center_axis',(-1.4081690688991E-16,0.,-1.));
#115103=DIRECTION('ref_axis',(-1.,0.,1.4081690688991E-16));
#115104=DIRECTION('center_axis',(-1.4081690688991E-16,0.,-1.));
#115105=DIRECTION('ref_axis',(-1.,0.,1.4081690688991E-16));
#115106=DIRECTION('center_axis',(-1.4081690688991E-16,0.,-1.));
#115107=DIRECTION('ref_axis',(-1.,0.,1.4081690688991E-16));
#115108=DIRECTION('',(0.994521895368273,-0.104528463267661,-1.40045497140051E-16));
#115109=DIRECTION('center_axis',(1.4081690688991E-16,0.,1.));
#115110=DIRECTION('ref_axis',(1.,0.,-1.4081690688991E-16));
#115111=DIRECTION('',(-0.489077884775286,0.103961598321231,0.866022406579776));
#115112=DIRECTION('center_axis',(1.4081690688991E-16,0.,1.));
#115113=DIRECTION('ref_axis',(-1.,1.59872115546023E-14,1.40816906889911E-16));
#115114=DIRECTION('',(0.497266609935035,-0.0522600224406424,-0.866022406579773));
#115115=DIRECTION('center_axis',(-1.4081690688991E-16,0.,-1.));
#115116=DIRECTION('ref_axis',(-1.,0.,1.40816906889911E-16));
#115117=DIRECTION('center_axis',(-1.4081690688991E-16,0.,-1.));
#115118=DIRECTION('ref_axis',(-1.,0.,1.4081690688991E-16));
#115119=DIRECTION('',(-0.978147600733804,0.207911690817766,1.37739719617121E-16));
#115120=DIRECTION('center_axis',(1.4081690688991E-16,0.,1.));
#115121=DIRECTION('ref_axis',(-1.,2.1316282072803E-14,1.4081690688991E-16));
#115122=DIRECTION('',(0.994521895368273,-0.104528463267661,-1.40045497140051E-16));
#115123=DIRECTION('center_axis',(-1.4081690688991E-16,0.,-1.));
#115124=DIRECTION('ref_axis',(-1.,0.,1.4081690688991E-16));
#115125=DIRECTION('center_axis',(-1.4081690688991E-16,0.,-1.));
#115126=DIRECTION('ref_axis',(1.,0.,-1.4081690688991E-16));
#115127=DIRECTION('',(-0.489079645219224,0.103952356682314,-0.866022521746652));
#115128=DIRECTION('center_axis',(-1.4081690688991E-16,0.,-1.));
#115129=DIRECTION('ref_axis',(-1.,0.,1.4081690688991E-16));
#115130=DIRECTION('center_axis',(-1.4081690688991E-16,0.,-1.));
#115131=DIRECTION('ref_axis',(-1.,0.,1.4081690688991E-16));
#115132=DIRECTION('center_axis',(-1.4081690688991E-16,0.,-1.));
#115133=DIRECTION('ref_axis',(-1.,0.,1.4081690688991E-16));
#115134=DIRECTION('',(0.497265428393238,-0.0522693557686635,0.866022521746645));
#115135=DIRECTION('center_axis',(-1.4081690688991E-16,0.,-1.));
#115136=DIRECTION('ref_axis',(-1.,0.,1.40816906889911E-16));
#115137=DIRECTION('',(-0.978147600733804,0.207911690817766,1.37739719617121E-16));
#115138=DIRECTION('center_axis',(1.4081690688991E-16,0.,1.));
#115139=DIRECTION('ref_axis',(-1.,2.57571741713036E-14,1.4081690688991E-16));
#115140=DIRECTION('',(0.994521895368273,-0.104528463267661,-1.40045497140051E-16));
#115141=DIRECTION('center_axis',(-1.4081690688991E-16,0.,-1.));
#115142=DIRECTION('ref_axis',(-1.,0.,1.17174841180864E-16));
#115143=DIRECTION('center_axis',(0.20686470343119,0.978369559222114,7.8645720103081E-6));
#115144=DIRECTION('ref_axis',(1.93871496019889E-7,7.99745532505487E-6,-0.999999999968001));
#115145=DIRECTION('center_axis',(-0.105592796389228,-0.994409453539563,
7.86457228715899E-6));
#115146=DIRECTION('ref_axis',(0.843303350210933,-0.0895515687886337,-0.529924500330482));
#115147=DIRECTION('center_axis',(-1.4081690688991E-16,0.,-1.));
#115148=DIRECTION('ref_axis',(-1.,0.,1.13676889660403E-16));
#115149=DIRECTION('center_axis',(0.206909324620437,0.978360123517741,-9.77058714809604E-6));
#115150=DIRECTION('ref_axis',(0.855713599898024,-0.180976161286533,-0.484769908302439));
#115151=DIRECTION('center_axis',(-0.105547443284143,-0.99441426836139,-9.7705161524926E-6));
#115152=DIRECTION('ref_axis',(0.86976418494061,-0.0923122812912277,-0.484756336026055));
#115153=DIRECTION('center_axis',(-1.4081690688991E-16,0.,-1.));
#115154=DIRECTION('ref_axis',(-1.,0.,1.15974593313694E-16));
#115155=DIRECTION('center_axis',(-0.210452521944373,-0.977604079204551,
1.81624797413716E-5));
#115156=DIRECTION('ref_axis',(0.845868804767752,-0.182084057578221,0.501349539838848));
#115157=DIRECTION('center_axis',(0.101944049587634,0.99479013385986,1.81316452525535E-5));
#115158=DIRECTION('ref_axis',(0.862463698455125,-0.0883925913422159,0.4983403642521));
#115159=DIRECTION('center_axis',(-1.4081690688991E-16,0.,-1.));
#115160=DIRECTION('ref_axis',(-1.,0.,1.16261524579732E-16));
#115161=DIRECTION('center_axis',(-0.210465731282001,-0.977601235480962,
1.84940588659675E-5));
#115162=DIRECTION('ref_axis',(0.847560772124303,-0.182479018596253,-0.498339387694976));
#115163=DIRECTION('center_axis',(0.101930608471476,0.994791511178816,1.85257108169065E-5));
#115164=DIRECTION('ref_axis',(0.860739767465406,-0.0881857549145489,-0.501348506862991));
#115165=DIRECTION('center_axis',(-1.4081690688991E-16,0.,-1.));
#115166=DIRECTION('ref_axis',(-1.,0.,1.40816906889911E-16));
#115167=DIRECTION('center_axis',(-1.4081690688991E-16,0.,-1.));
#115168=DIRECTION('ref_axis',(-1.,0.,1.4081690688991E-16));
#115169=DIRECTION('',(-0.994521895368273,0.104528463267661,1.40045497140051E-16));
#115170=DIRECTION('center_axis',(-1.4081690688991E-16,0.,-1.));
#115171=DIRECTION('ref_axis',(-1.,0.,1.4081690688991E-16));
#115172=DIRECTION('center_axis',(-1.4081690688991E-16,0.,-1.));
#115173=DIRECTION('ref_axis',(-1.,0.,1.4081690688991E-16));
#115174=DIRECTION('center_axis',(-1.4081690688991E-16,0.,-1.));
#115175=DIRECTION('ref_axis',(-1.,0.,1.4081690688991E-16));
#115176=DIRECTION('',(1.,0.,-1.40816906889911E-16));
#115177=DIRECTION('center_axis',(1.4081690688991E-16,0.,1.));
#115178=DIRECTION('ref_axis',(1.,0.,-1.4081690688991E-16));
#115179=DIRECTION('',(-0.49726561106078,0.0522695260941912,0.866022406579783));
#115180=DIRECTION('center_axis',(1.4081690688991E-16,0.,1.));
#115181=DIRECTION('ref_axis',(-1.,6.21724893790088E-15,1.40816906889911E-16));
#115182=DIRECTION('',(0.500005191251985,4.77800116551749E-6,-0.866022406579782));
#115183=DIRECTION('center_axis',(-1.4081690688991E-16,0.,-1.));
#115184=DIRECTION('ref_axis',(-1.,0.,1.40816906889911E-16));
#115185=DIRECTION('center_axis',(-1.4081690688991E-16,0.,-1.));
#115186=DIRECTION('ref_axis',(-1.,0.,1.4081690688991E-16));
#115187=DIRECTION('',(-0.994521895368273,0.104528463267661,1.40045497140051E-16));
#115188=DIRECTION('center_axis',(1.4081690688991E-16,0.,1.));
#115189=DIRECTION('ref_axis',(-1.,1.33226762955019E-14,1.4081690688991E-16));
#115190=DIRECTION('',(1.,0.,-1.40816906889911E-16));
#115191=DIRECTION('center_axis',(-1.4081690688991E-16,0.,-1.));
#115192=DIRECTION('ref_axis',(-1.,0.,1.4081690688991E-16));
#115193=DIRECTION('center_axis',(-1.4081690688991E-16,0.,-1.));
#115194=DIRECTION('ref_axis',(1.,0.,-1.4081690688991E-16));
#115195=DIRECTION('',(-0.497266395846527,0.0522601510654385,-0.866022521746648));
#115196=DIRECTION('center_axis',(-1.4081690688991E-16,0.,-1.));
#115197=DIRECTION('ref_axis',(-1.,0.,1.4081690688991E-16));
#115198=DIRECTION('center_axis',(-1.4081690688991E-16,0.,-1.));
#115199=DIRECTION('ref_axis',(-1.,0.,1.4081690688991E-16));
#115200=DIRECTION('center_axis',(-1.4081690688991E-16,0.,-1.));
#115201=DIRECTION('ref_axis',(-1.,0.,1.4081690688991E-16));
#115202=DIRECTION('',(0.500004991781227,-4.62770265276808E-6,0.866022521746657));
#115203=DIRECTION('center_axis',(-1.4081690688991E-16,0.,-1.));
#115204=DIRECTION('ref_axis',(-1.,0.,1.40816906889911E-16));
#115205=DIRECTION('',(-0.994521895368273,0.104528463267661,1.40045497140051E-16));
#115206=DIRECTION('center_axis',(1.4081690688991E-16,0.,1.));
#115207=DIRECTION('ref_axis',(-1.,1.86517468137026E-14,1.4081690688991E-16));
#115208=DIRECTION('',(1.,0.,-1.40816906889911E-16));
#115209=DIRECTION('center_axis',(-1.4081690688991E-16,0.,-1.));
#115210=DIRECTION('ref_axis',(-1.,0.,1.17174841180864E-16));
#115211=DIRECTION('center_axis',(0.103464010407829,0.994633197962182,7.86457202866399E-6));
#115212=DIRECTION('ref_axis',(-6.43152314414483E-7,7.97390954032807E-6,
-0.999999999968002));
#115213=DIRECTION('center_axis',(-0.00107025596492904,-0.999999427244995,
7.86457228903988E-6));
#115214=DIRECTION('ref_axis',(0.848044334090885,-0.000911792658859396,-0.529924500330466));
#115215=DIRECTION('center_axis',(-1.4081690688991E-16,0.,-1.));
#115216=DIRECTION('ref_axis',(-1.,0.,1.13676889660403E-16));
#115217=DIRECTION('center_axis',(0.103509373457831,0.994628478131862,-9.77058613603921E-6));
#115218=DIRECTION('ref_axis',(0.869943071289075,-0.0905383273444945,-0.484769908304747));
#115219=DIRECTION('center_axis',(-0.00102464802304199,-0.999999475000345,
-9.77051628002253E-6));
#115220=DIRECTION('ref_axis',(0.874648786634557,-0.000891471298430306,-0.484756336026278));
#115221=DIRECTION('center_axis',(-1.4081690688991E-16,0.,-1.));
#115222=DIRECTION('ref_axis',(-1.,0.,1.15974593313694E-16));
#115223=DIRECTION('center_axis',(-0.10711218892573,-0.994246940479911,1.8162479773676E-5));
#115224=DIRECTION('ref_axis',(0.860268013676508,-0.0926692157708133,0.50134953983573));
#115225=DIRECTION('center_axis',(-0.0025982945487866,0.999996624262643,
1.81316452254577E-5));
#115226=DIRECTION('ref_axis',(0.866978573812158,0.00224363754549588,0.49834036425038));
#115227=DIRECTION('center_axis',(-1.4081690688991E-16,0.,-1.));
#115228=DIRECTION('ref_axis',(-1.,0.,1.16261524579732E-16));
#115229=DIRECTION('center_axis',(-0.1071256231494,-0.994245493086503,1.84940621084383E-5));
#115230=DIRECTION('ref_axis',(0.861991996926058,-0.0928851544032616,-0.498339387693677));
#115231=DIRECTION('center_axis',(-0.00261180600216756,0.999996589057285,
1.85257107824588E-5));
#115232=DIRECTION('ref_axis',(0.865242466405598,0.00226914104443776,-0.501348506856535));
#115233=DIRECTION('center_axis',(-1.4081690688991E-16,0.,-1.));
#115234=DIRECTION('ref_axis',(-1.,0.,1.40816906889911E-16));
#115235=DIRECTION('center_axis',(-1.4081690688991E-16,0.,-1.));
#115236=DIRECTION('ref_axis',(-1.,0.,1.4081690688991E-16));
#115237=DIRECTION('',(-1.,0.,1.40816906889911E-16));
#115238=DIRECTION('center_axis',(-1.4081690688991E-16,0.,-1.));
#115239=DIRECTION('ref_axis',(-1.,0.,1.4081690688991E-16));
#115240=DIRECTION('center_axis',(-1.4081690688991E-16,0.,-1.));
#115241=DIRECTION('ref_axis',(-1.,0.,1.4081690688991E-16));
#115242=DIRECTION('center_axis',(-1.4081690688991E-16,0.,-1.));
#115243=DIRECTION('ref_axis',(-1.,0.,1.4081690688991E-16));
#115244=DIRECTION('',(0.994521895368274,0.104528463267647,-1.40045497140052E-16));
#115245=DIRECTION('center_axis',(1.4081690688991E-16,0.,1.));
#115246=DIRECTION('ref_axis',(1.,0.,-1.4081690688991E-16));
#115247=DIRECTION('',(-0.500005191251985,4.77800116551749E-6,0.866022406579782));
#115248=DIRECTION('center_axis',(1.4081690688991E-16,0.,1.));
#115249=DIRECTION('ref_axis',(-1.,0.,1.40816906889911E-16));
#115250=DIRECTION('',(0.49726561106078,0.0522695260941878,-0.866022406579783));
#115251=DIRECTION('center_axis',(-1.4081690688991E-16,0.,-1.));
#115252=DIRECTION('ref_axis',(-1.,0.,1.40816906889911E-16));
#115253=DIRECTION('center_axis',(-1.4081690688991E-16,0.,-1.));
#115254=DIRECTION('ref_axis',(-1.,0.,1.4081690688991E-16));
#115255=DIRECTION('',(-1.,0.,1.40816906889911E-16));
#115256=DIRECTION('center_axis',(1.4081690688991E-16,0.,1.));
#115257=DIRECTION('ref_axis',(-1.,0.,1.4081690688991E-16));
#115258=DIRECTION('',(0.994521895368274,0.104528463267647,-1.40045497140052E-16));
#115259=DIRECTION('center_axis',(-1.4081690688991E-16,0.,-1.));
#115260=DIRECTION('ref_axis',(-1.,0.,1.4081690688991E-16));
#115261=DIRECTION('center_axis',(-1.4081690688991E-16,0.,-1.));
#115262=DIRECTION('ref_axis',(1.,0.,-1.4081690688991E-16));
#115263=DIRECTION('',(-0.500004991781227,-4.62770265276808E-6,-0.866022521746657));
#115264=DIRECTION('center_axis',(-1.4081690688991E-16,0.,-1.));
#115265=DIRECTION('ref_axis',(-1.,0.,1.4081690688991E-16));
#115266=DIRECTION('center_axis',(-1.4081690688991E-16,0.,-1.));
#115267=DIRECTION('ref_axis',(-1.,0.,1.4081690688991E-16));
#115268=DIRECTION('center_axis',(-1.4081690688991E-16,0.,-1.));
#115269=DIRECTION('ref_axis',(-1.,0.,1.4081690688991E-16));
#115270=DIRECTION('',(0.497266395846506,0.0522601510654325,0.86602252174666));
#115271=DIRECTION('center_axis',(-1.4081690688991E-16,0.,-1.));
#115272=DIRECTION('ref_axis',(-1.,0.,1.40816906889911E-16));
#115273=DIRECTION('',(-1.,0.,1.40816906889911E-16));
#115274=DIRECTION('center_axis',(1.4081690688991E-16,0.,1.));
#115275=DIRECTION('ref_axis',(-1.,0.,1.4081690688991E-16));
#115276=DIRECTION('',(0.994521895368274,0.104528463267647,-1.40045497140052E-16));
#115277=DIRECTION('center_axis',(-1.4081690688991E-16,0.,-1.));
#115278=DIRECTION('ref_axis',(-1.,0.,1.17174841180864E-16));
#115279=DIRECTION('center_axis',(-0.00107025596477632,0.999999427244995,
7.86457201352231E-6));
#115280=DIRECTION('ref_axis',(-1.47312954961581E-6,7.86299989115223E-6,
-0.999999999968002));
#115281=DIRECTION('center_axis',(0.103464010407674,-0.994633197962198,7.86457229252233E-6));
#115282=DIRECTION('ref_axis',(0.843493966781838,0.0877379732620788,-0.529924500330474));
#115283=DIRECTION('center_axis',(-1.4081690688991E-16,0.,-1.));
#115284=DIRECTION('ref_axis',(-1.,0.,1.13676889660403E-16));
#115285=DIRECTION('center_axis',(-0.00102464806169058,0.999999475000305,
-9.77058600455096E-6));
#115286=DIRECTION('ref_axis',(0.87464126434622,0.000891463458123506,-0.484769908302639));
#115287=DIRECTION('center_axis',(0.103509373496272,-0.994628478127862,-9.77051629371499E-6));
#115288=DIRECTION('ref_axis',(0.869950553189069,0.0905391058403209,-0.484756336028388));
#115289=DIRECTION('center_axis',(-1.4081690688991E-16,0.,-1.));
#115290=DIRECTION('ref_axis',(-1.,0.,1.15974593313694E-16));
#115291=DIRECTION('center_axis',(-0.0025983123505633,-0.999996624215829,
1.81624797797147E-5));
#115292=DIRECTION('ref_axis',(0.865241946200303,-0.00223907064277699,0.501349539840388));
#115293=DIRECTION('center_axis',(-0.107112171226437,0.994246942387253,1.81316453094968E-5));
#115294=DIRECTION('ref_axis',(0.861994650482721,0.0928552846704071,0.49834036425715));
#115295=DIRECTION('center_axis',(-1.4081690688991E-16,0.,-1.));
#115296=DIRECTION('ref_axis',(-1.,0.,1.16261524579732E-16));
#115297=DIRECTION('center_axis',(-0.00261182427503963,-0.999996589010146,
1.84940601579397E-5));
#115298=DIRECTION('ref_axis',(0.866979057020118,-0.00227362102098959,-0.498339387702758));
#115299=DIRECTION('center_axis',(-0.107125604985124,0.994245495043035,1.85257064812721E-5));
#115300=DIRECTION('ref_axis',(0.860265387813178,0.092699175819291,-0.501348506862309));
#115301=DIRECTION('center_axis',(-1.4081690688991E-16,0.,-1.));
#115302=DIRECTION('ref_axis',(-1.,0.,1.40816906889911E-16));
#115303=DIRECTION('center_axis',(-1.4081690688991E-16,0.,-1.));
#115304=DIRECTION('ref_axis',(-1.,0.,1.4081690688991E-16));
#115305=DIRECTION('',(-0.994521895368274,-0.104528463267647,1.40045497140052E-16));
#115306=DIRECTION('center_axis',(-1.4081690688991E-16,0.,-1.));
#115307=DIRECTION('ref_axis',(-1.,0.,1.4081690688991E-16));
#115308=DIRECTION('center_axis',(-1.4081690688991E-16,0.,-1.));
#115309=DIRECTION('ref_axis',(-1.,0.,1.4081690688991E-16));
#115310=DIRECTION('center_axis',(-1.4081690688991E-16,0.,-1.));
#115311=DIRECTION('ref_axis',(-1.,0.,1.4081690688991E-16));
#115312=DIRECTION('',(0.978147600733807,0.207911690817753,-1.37739719617122E-16));
#115313=DIRECTION('center_axis',(1.4081690688991E-16,0.,1.));
#115314=DIRECTION('ref_axis',(1.,0.,-1.4081690688991E-16));
#115315=DIRECTION('',(-0.497266609935035,-0.0522600224406356,0.866022406579773));
#115316=DIRECTION('center_axis',(1.4081690688991E-16,0.,1.));
#115317=DIRECTION('ref_axis',(-1.,0.,1.40816906889911E-16));
#115318=DIRECTION('',(0.489077884775245,0.103961598321228,-0.8660224065798));
#115319=DIRECTION('center_axis',(-1.4081690688991E-16,0.,-1.));
#115320=DIRECTION('ref_axis',(-1.,0.,1.40816906889911E-16));
#115321=DIRECTION('center_axis',(-1.4081690688991E-16,0.,-1.));
#115322=DIRECTION('ref_axis',(-1.,0.,1.4081690688991E-16));
#115323=DIRECTION('',(-0.994521895368274,-0.104528463267647,1.40045497140052E-16));
#115324=DIRECTION('center_axis',(1.4081690688991E-16,0.,1.));
#115325=DIRECTION('ref_axis',(-1.,0.,1.4081690688991E-16));
#115326=DIRECTION('',(0.978147600733807,0.207911690817753,-1.37739719617122E-16));
#115327=DIRECTION('center_axis',(-1.4081690688991E-16,0.,-1.));
#115328=DIRECTION('ref_axis',(-1.,0.,1.4081690688991E-16));
#115329=DIRECTION('center_axis',(-1.4081690688991E-16,0.,-1.));
#115330=DIRECTION('ref_axis',(1.,0.,-1.4081690688991E-16));
#115331=DIRECTION('',(-0.497265428393217,-0.0522693557686642,-0.866022521746657));
#115332=DIRECTION('center_axis',(-1.4081690688991E-16,0.,-1.));
#115333=DIRECTION('ref_axis',(-1.,0.,1.4081690688991E-16));
#115334=DIRECTION('center_axis',(-1.4081690688991E-16,0.,-1.));
#115335=DIRECTION('ref_axis',(-1.,0.,1.4081690688991E-16));
#115336=DIRECTION('center_axis',(-1.4081690688991E-16,0.,-1.));
#115337=DIRECTION('ref_axis',(-1.,0.,1.4081690688991E-16));
#115338=DIRECTION('',(0.489079645219225,0.1039523566823,0.866022521746653));
#115339=DIRECTION('center_axis',(-1.4081690688991E-16,0.,-1.));
#115340=DIRECTION('ref_axis',(-1.,0.,1.40816906889911E-16));
#115341=DIRECTION('',(-0.994521895368274,-0.104528463267647,1.40045497140052E-16));
#115342=DIRECTION('center_axis',(1.4081690688991E-16,0.,1.));
#115343=DIRECTION('ref_axis',(-1.,0.,1.4081690688991E-16));
#115344=DIRECTION('',(0.978147600733807,0.207911690817753,-1.37739719617122E-16));
#115345=DIRECTION('center_axis',(-1.4081690688991E-16,0.,-1.));
#115346=DIRECTION('ref_axis',(-1.,0.,1.17174841180864E-16));
#115347=DIRECTION('center_axis',(-0.105592796389083,0.994409453539578,7.86457203806509E-6));
#115348=DIRECTION('ref_axis',(-2.28696684648491E-6,7.66594161629955E-6,
-0.999999999968002));
#115349=DIRECTION('center_axis',(0.206864703430992,-0.978369559222156,7.86457234781368E-6));
#115350=DIRECTION('ref_axis',(0.829702103060314,0.175426463587569,-0.529924500330426));
#115351=DIRECTION('center_axis',(-1.4081690688991E-16,0.,-1.));
#115352=DIRECTION('ref_axis',(-1.,0.,1.13676889660403E-16));
#115353=DIRECTION('center_axis',(-0.105547443321288,0.994414268357446,-9.77058366484796E-6));
#115354=DIRECTION('ref_axis',(0.869756704679168,0.0923114872005142,-0.484769908303376));
#115355=DIRECTION('center_axis',(0.206909324660093,-0.978360123509355,-9.77051398001622E-6));
#115356=DIRECTION('ref_axis',(0.855720959435109,0.180977717588947,-0.484756336028474));
#115357=DIRECTION('center_axis',(-1.4081690688991E-16,0.,-1.));
#115358=DIRECTION('ref_axis',(-1.,0.,1.15974593313694E-16));
#115359=DIRECTION('center_axis',(0.10194403187845,-0.994790135674098,1.8162479803541E-5));
#115360=DIRECTION('ref_axis',(0.860736106899776,0.088215606211404,0.501349539841987));
#115361=DIRECTION('center_axis',(-0.210452504541383,0.97760408295153,1.81316452253489E-5));
#115362=DIRECTION('ref_axis',(0.847566533385468,0.182449589865907,0.498340364251887));
#115363=DIRECTION('center_axis',(-1.4081690688991E-16,0.,-1.));
#115364=DIRECTION('ref_axis',(-1.,0.,1.16261524579732E-16));
#115365=DIRECTION('center_axis',(0.101930590294196,-0.994791513041927,1.84940609616093E-5));
#115366=DIRECTION('ref_axis',(0.862467313149233,0.088362822628976,-0.498339387692949));
#115367=DIRECTION('center_axis',(-0.210465713418174,0.977601239326228,1.8525709565287E-5));
#115368=DIRECTION('ref_axis',(0.845863061613277,0.182113579025382,-0.501348506862022));
#115369=DIRECTION('center_axis',(-1.4081690688991E-16,0.,-1.));
#115370=DIRECTION('ref_axis',(-1.,0.,1.40816906889911E-16));
#115371=DIRECTION('center_axis',(-1.4081690688991E-16,0.,-1.));
#115372=DIRECTION('ref_axis',(-1.,0.,1.4081690688991E-16));
#115373=DIRECTION('',(-0.978147600733807,-0.207911690817753,1.37739719617122E-16));
#115374=DIRECTION('center_axis',(-1.4081690688991E-16,0.,-1.));
#115375=DIRECTION('ref_axis',(-1.,0.,1.4081690688991E-16));
#115376=DIRECTION('center_axis',(-1.4081690688991E-16,0.,-1.));
#115377=DIRECTION('ref_axis',(-1.,0.,1.4081690688991E-16));
#115378=DIRECTION('center_axis',(-1.4081690688991E-16,0.,-1.));
#115379=DIRECTION('ref_axis',(-1.,0.,1.4081690688991E-16));
#115380=DIRECTION('',(0.951056516295155,0.309016994374942,-1.33924836902178E-16));
#115381=DIRECTION('center_axis',(1.4081690688991E-16,0.,1.));
#115382=DIRECTION('ref_axis',(1.,0.,-1.4081690688991E-16));
#115383=DIRECTION('',(-0.489079871579893,-0.103952251140478,0.866022406579773));
#115384=DIRECTION('center_axis',(1.4081690688991E-16,0.,1.));
#115385=DIRECTION('ref_axis',(-1.,0.,1.40816906889911E-16));
#115386=DIRECTION('',(0.475531718838024,0.154514645521709,-0.866022406579792));
#115387=DIRECTION('center_axis',(-1.4081690688991E-16,0.,-1.));
#115388=DIRECTION('ref_axis',(-1.,0.,1.40816906889911E-16));
#115389=DIRECTION('center_axis',(-1.4081690688991E-16,0.,-1.));
#115390=DIRECTION('ref_axis',(-1.,0.,1.4081690688991E-16));
#115391=DIRECTION('',(-0.978147600733807,-0.207911690817753,1.37739719617122E-16));
#115392=DIRECTION('center_axis',(1.4081690688991E-16,0.,1.));
#115393=DIRECTION('ref_axis',(-1.,0.,1.4081690688991E-16));
#115394=DIRECTION('',(0.951056516295155,0.309016994374942,-1.33924836902177E-16));
#115395=DIRECTION('center_axis',(-1.4081690688991E-16,0.,-1.));
#115396=DIRECTION('ref_axis',(-1.,0.,1.4081690688991E-16));
#115397=DIRECTION('center_axis',(-1.4081690688991E-16,0.,-1.));
#115398=DIRECTION('ref_axis',(1.,0.,-1.4081690688991E-16));
#115399=DIRECTION('',(-0.489077720912262,-0.103961409834802,-0.86602252174665));
#115400=DIRECTION('center_axis',(-1.4081690688991E-16,0.,-1.));
#115401=DIRECTION('ref_axis',(-1.,0.,1.4081690688991E-16));
#115402=DIRECTION('center_axis',(-1.4081690688991E-16,0.,-1.));
#115403=DIRECTION('ref_axis',(-1.,0.,1.4081690688991E-16));
#115404=DIRECTION('center_axis',(-1.4081690688991E-16,0.,-1.));
#115405=DIRECTION('ref_axis',(-1.,0.,1.4081690688991E-16));
#115406=DIRECTION('',(0.475534435652402,0.154505638525938,0.86602252174666));
#115407=DIRECTION('center_axis',(-1.4081690688991E-16,0.,-1.));
#115408=DIRECTION('ref_axis',(-1.,0.,1.40816906889911E-16));
#115409=DIRECTION('',(-0.978147600733807,-0.207911690817753,1.37739719617122E-16));
#115410=DIRECTION('center_axis',(1.4081690688991E-16,0.,1.));
#115411=DIRECTION('ref_axis',(-1.,0.,1.4081690688991E-16));
#115412=DIRECTION('',(0.951056516295155,0.309016994374942,-1.33924836902178E-16));
#115413=DIRECTION('center_axis',(-1.4081690688991E-16,0.,-1.));
#115414=DIRECTION('ref_axis',(-1.,0.,1.17174841180864E-16));
#115415=DIRECTION('center_axis',(-0.208958440039409,0.977924521767629,7.86457200610629E-6));
#115416=DIRECTION('ref_axis',(-3.07574767837473E-6,7.38489362573465E-6,
-0.999999999968002));
#115417=DIRECTION('center_axis',(0.307998943474345,-0.951386698854275,7.86457233122683E-6));
#115418=DIRECTION('ref_axis',(0.806819849471267,0.261192944867712,-0.529924500330468));
#115419=DIRECTION('center_axis',(-1.4081690688991E-16,0.,-1.));
#115420=DIRECTION('ref_axis',(-1.,0.,1.13676889660403E-16));
#115421=DIRECTION('center_axis',(-0.208913838706489,0.977934050895793,-9.77058458900962E-6));
#115422=DIRECTION('ref_axis',(0.855342908549112,0.182720126972052,-0.4847699083009));
#115423=DIRECTION('center_axis',(0.308042333962515,-0.951372650642987,-9.77051510954378E-6));
#115424=DIRECTION('ref_axis',(0.832115907779389,0.269433499591945,-0.484756336026793));
#115425=DIRECTION('center_axis',(-1.4081690688991E-16,0.,-1.));
#115426=DIRECTION('ref_axis',(-1.,0.,1.15974593313694E-16));
#115427=DIRECTION('center_axis',(0.205369455961064,-0.978684518232704,1.81624798317175E-5));
#115428=DIRECTION('ref_axis',(0.846799862697162,0.177703774424654,0.501349539833536));
#115429=DIRECTION('center_axis',(-0.311487076176632,0.95025038860617,1.8131645292547E-5));
#115430=DIRECTION('ref_axis',(0.82385229998436,0.270044939175662,0.498340364245255));
#115431=DIRECTION('center_axis',(-1.4081690688991E-16,0.,-1.));
#115432=DIRECTION('ref_axis',(-1.,0.,1.16261524579732E-16));
#115433=DIRECTION('center_axis',(0.205356231986127,-0.978687293083153,1.84940623151564E-5));
#115434=DIRECTION('ref_axis',(0.848506196903301,0.178031144702363,-0.49833938769945));
#115435=DIRECTION('center_axis',(-0.311499915451504,0.95024617985578,1.85257141175826E-5));
#115436=DIRECTION('ref_axis',(0.822193282701921,0.269532707749929,-0.501348506862074));
#115437=DIRECTION('center_axis',(-1.4081690688991E-16,0.,-1.));
#115438=DIRECTION('ref_axis',(-1.,0.,1.40816906889911E-16));
#115439=DIRECTION('center_axis',(-1.4081690688991E-16,0.,-1.));
#115440=DIRECTION('ref_axis',(-1.,0.,1.4081690688991E-16));
#115441=DIRECTION('',(-0.951056516295155,-0.309016994374942,1.33924836902178E-16));
#115442=DIRECTION('center_axis',(-1.4081690688991E-16,0.,-1.));
#115443=DIRECTION('ref_axis',(-1.,0.,1.4081690688991E-16));
#115444=DIRECTION('center_axis',(-1.4081690688991E-16,0.,-1.));
#115445=DIRECTION('ref_axis',(-1.,0.,1.4081690688991E-16));
#115446=DIRECTION('center_axis',(-1.4081690688991E-16,0.,-1.));
#115447=DIRECTION('ref_axis',(-1.,0.,1.4081690688991E-16));
#115448=DIRECTION('',(0.913545457642603,0.406736643075795,-1.28642645648559E-16));
#115449=DIRECTION('center_axis',(1.4081690688991E-16,0.,1.));
#115450=DIRECTION('ref_axis',(1.,0.,-1.4081690688991E-16));
#115451=DIRECTION('',(-0.475534671805141,-0.154505557223416,0.866022406579794));
#115452=DIRECTION('center_axis',(1.4081690688991E-16,0.,1.));
#115453=DIRECTION('ref_axis',(-1.,0.,1.40816906889911E-16));
#115454=DIRECTION('',(0.456775527877798,0.20337479793158,-0.866022406579788));
#115455=DIRECTION('center_axis',(-1.4081690688991E-16,0.,-1.));
#115456=DIRECTION('ref_axis',(-1.,0.,1.40816906889911E-16));
#115457=DIRECTION('center_axis',(-1.4081690688991E-16,0.,-1.));
#115458=DIRECTION('ref_axis',(-1.,0.,1.4081690688991E-16));
#115459=DIRECTION('',(-0.951056516295155,-0.309016994374942,1.33924836902178E-16));
#115460=DIRECTION('center_axis',(1.4081690688991E-16,0.,1.));
#115461=DIRECTION('ref_axis',(-1.,0.,1.4081690688991E-16));
#115462=DIRECTION('',(0.913545457642603,0.406736643075795,-1.28642645648559E-16));
#115463=DIRECTION('center_axis',(-1.4081690688991E-16,0.,-1.));
#115464=DIRECTION('ref_axis',(-1.,0.,1.4081690688991E-16));
#115465=DIRECTION('center_axis',(-1.4081690688991E-16,0.,-1.));
#115466=DIRECTION('ref_axis',(1.,0.,-1.4081690688991E-16));
#115467=DIRECTION('',(-0.47553157557486,-0.154514440939468,-0.866022521746666));
#115468=DIRECTION('center_axis',(-1.4081690688991E-16,0.,-1.));
#115469=DIRECTION('ref_axis',(-1.,0.,1.4081690688991E-16));
#115470=DIRECTION('center_axis',(-1.4081690688991E-16,0.,-1.));
#115471=DIRECTION('ref_axis',(-1.,0.,1.4081690688991E-16));
#115472=DIRECTION('center_axis',(-1.4081690688991E-16,0.,-1.));
#115473=DIRECTION('ref_axis',(-1.,0.,1.4081690688991E-16));
#115474=DIRECTION('',(0.456779171296622,0.203366124261496,0.866022521746652));
#115475=DIRECTION('center_axis',(-1.4081690688991E-16,0.,-1.));
#115476=DIRECTION('ref_axis',(-1.,0.,1.40816906889911E-16));
#115477=DIRECTION('',(-0.951056516295155,-0.309016994374942,1.33924836902178E-16));
#115478=DIRECTION('center_axis',(1.4081690688991E-16,0.,1.));
#115479=DIRECTION('ref_axis',(-1.,0.,1.4081690688991E-16));
#115480=DIRECTION('',(0.913545457642603,0.406736643075795,-1.28642645648559E-16));
#115481=DIRECTION('center_axis',(-1.4081690688991E-16,0.,-1.));
#115482=DIRECTION('ref_axis',(-1.,0.,1.17174841180864E-16));
#115483=DIRECTION('center_axis',(-0.31003469129331,0.950725244291331,7.86457199748011E-6));
#115484=DIRECTION('ref_axis',(-3.83083002565344E-6,7.02293521153946E-6,
-0.999999999968002));
#115485=DIRECTION('center_axis',(0.405758682640086,-0.91398024672327,7.8645722503889E-6));
#115486=DIRECTION('ref_axis',(0.775097908773512,0.3440977415858,-0.529924500330454));
#115487=DIRECTION('center_axis',(-1.4081690688991E-16,0.,-1.));
#115488=DIRECTION('ref_axis',(-1.,0.,1.13676889660403E-16));
#115489=DIRECTION('center_axis',(-0.309991330354646,0.950739383327257,-9.77058136445211E-6));
#115490=DIRECTION('ref_axis',(0.83155779651886,0.27112684679551,-0.484769908302303));
#115491=DIRECTION('center_axis',(0.405800366992456,-0.913961739928606,-9.77051546410327E-6));
#115492=DIRECTION('ref_axis',(0.79939402010551,0.354937311790544,-0.484756336027137));
#115493=DIRECTION('center_axis',(-1.4081690688991E-16,0.,-1.));
#115494=DIRECTION('ref_axis',(-1.,0.,1.15974593313694E-16));
#115495=DIRECTION('center_axis',(0.306544809308013,-0.951856228406601,1.8162479602898E-5));
#115496=DIRECTION('ref_axis',(0.823585901985266,0.265244982896496,0.501349539841568));
#115497=DIRECTION('center_axis',(-0.409108930222373,0.91248555215058,1.81316452010363E-5));
#115498=DIRECTION('ref_axis',(0.791111768373646,0.354681619618225,0.49834036425491));
#115499=DIRECTION('center_axis',(-1.4081690688991E-16,0.,-1.));
#115500=DIRECTION('ref_axis',(-1.,0.,1.16261524579732E-16));
#115501=DIRECTION('center_axis',(0.306531947823564,-0.951860370338771,1.84940577497957E-5));
#115502=DIRECTION('ref_axis',(0.825248669208761,0.265748920300067,-0.498339387695291));
#115503=DIRECTION('center_axis',(-0.409121259232272,0.912480024384643,1.85257063074674E-5));
#115504=DIRECTION('ref_axis',(0.789515382129243,0.353998779724516,-0.501348506864107));
#115505=DIRECTION('center_axis',(-1.4081690688991E-16,0.,-1.));
#115506=DIRECTION('ref_axis',(-1.,0.,1.40816906889911E-16));
#115507=DIRECTION('center_axis',(-1.4081690688991E-16,0.,-1.));
#115508=DIRECTION('ref_axis',(-1.,0.,1.4081690688991E-16));
#115509=DIRECTION('',(-0.913545457642603,-0.406736643075795,1.28642645648559E-16));
#115510=DIRECTION('center_axis',(-1.4081690688991E-16,0.,-1.));
#115511=DIRECTION('ref_axis',(-1.,0.,1.4081690688991E-16));
#115512=DIRECTION('center_axis',(-1.4081690688991E-16,0.,-1.));
#115513=DIRECTION('ref_axis',(-1.,0.,1.4081690688991E-16));
#115514=DIRECTION('center_axis',(-1.4081690688991E-16,0.,-1.));
#115515=DIRECTION('ref_axis',(-1.,0.,1.4081690688991E-16));
#115516=DIRECTION('',(0.866025403784442,0.499999999999995,-1.21951018649011E-16));
#115517=DIRECTION('center_axis',(1.4081690688991E-16,0.,1.));
#115518=DIRECTION('ref_axis',(1.,0.,-1.4081690688991E-16));
#115519=DIRECTION('',(-0.456779414654131,-0.203366068089033,0.866022406579781));
#115520=DIRECTION('center_axis',(1.4081690688991E-16,0.,1.));
#115521=DIRECTION('ref_axis',(-1.,0.,1.40816906889911E-16));
#115522=DIRECTION('',(0.433014808647734,0.250006733496366,-0.866022406579785));
#115523=DIRECTION('center_axis',(-1.4081690688991E-16,0.,-1.));
#115524=DIRECTION('ref_axis',(-1.,0.,1.40816906889911E-16));
#115525=DIRECTION('center_axis',(-1.4081690688991E-16,0.,-1.));
#115526=DIRECTION('ref_axis',(-1.,0.,1.4081690688991E-16));
#115527=DIRECTION('',(-0.913545457642603,-0.406736643075795,1.28642645648559E-16));
#115528=DIRECTION('center_axis',(1.4081690688991E-16,0.,1.));
#115529=DIRECTION('ref_axis',(-1.,8.88178419700125E-16,1.4081690688991E-16));
#115530=DIRECTION('',(0.866025403784442,0.499999999999995,-1.21951018649011E-16));
#115531=DIRECTION('center_axis',(-1.4081690688991E-16,0.,-1.));
#115532=DIRECTION('ref_axis',(-1.,0.,1.4081690688991E-16));
#115533=DIRECTION('center_axis',(-1.4081690688991E-16,0.,-1.));
#115534=DIRECTION('ref_axis',(1.,0.,-1.4081690688991E-16));
#115535=DIRECTION('',(-0.456775406784116,-0.203374579494969,-0.866022521746663));
#115536=DIRECTION('center_axis',(-1.4081690688991E-16,0.,-1.));
#115537=DIRECTION('ref_axis',(-1.,0.,1.4081690688991E-16));
#115538=DIRECTION('center_axis',(-1.4081690688991E-16,0.,-1.));
#115539=DIRECTION('ref_axis',(-1.,0.,1.4081690688991E-16));
#115540=DIRECTION('center_axis',(-1.4081690688991E-16,0.,-1.));
#115541=DIRECTION('ref_axis',(-1.,0.,1.4081690688991E-16));
#115542=DIRECTION('',(0.433019338752908,0.24999848818253,0.86602252174666));
#115543=DIRECTION('center_axis',(-1.4081690688991E-16,0.,-1.));
#115544=DIRECTION('ref_axis',(-1.,0.,1.40816906889911E-16));
#115545=DIRECTION('',(-0.913545457642603,-0.406736643075795,1.28642645648559E-16));
#115546=DIRECTION('center_axis',(1.4081690688991E-16,0.,1.));
#115547=DIRECTION('ref_axis',(-1.,8.88178419700125E-16,1.4081690688991E-16));
#115548=DIRECTION('',(0.866025403784442,0.499999999999995,-1.21951018649011E-16));
#115549=DIRECTION('center_axis',(-1.4081690688991E-16,0.,-1.));
#115550=DIRECTION('ref_axis',(-1.,0.,1.17174841180864E-16));
#115551=DIRECTION('center_axis',(-0.40771413759047,0.913109622086531,7.86457197304048E-6));
#115552=DIRECTION('ref_axis',(-4.54394095516333E-6,6.58403203744326E-6,
-0.999999999968002));
#115553=DIRECTION('center_axis',(0.499072844768321,-0.866560035746517,7.86457228842995E-6));
#115554=DIRECTION('ref_axis',(0.734883833187592,0.423232531439894,-0.529924500330462));
#115555=DIRECTION('center_axis',(-1.4081690688991E-16,0.,-1.));
#115556=DIRECTION('ref_axis',(-1.,0.,1.13676889660403E-16));
#115557=DIRECTION('center_axis',(-0.407672492120574,0.913128216119038,-9.77058401182242E-6));
#115558=DIRECTION('ref_axis',(0.798661963254375,0.356563044147856,-0.484769908305663));
#115559=DIRECTION('center_axis',(0.499112366279568,-0.866537273134484,-9.77052188210463E-6));
#115560=DIRECTION('ref_axis',(0.757913804263745,0.436552356525934,-0.484756336026784));
#115561=DIRECTION('center_axis',(-1.4081690688991E-16,0.,-1.));
#115562=DIRECTION('ref_axis',(-1.,0.,1.15974593313694E-16));
#115563=DIRECTION('center_axis',(0.404361593575301,-0.914599202553428,1.81624797722619E-5));
#115564=DIRECTION('ref_axis',(0.791348561789598,0.349880111830676,0.501349539841106));
#115565=DIRECTION('center_axis',(-0.502248501217083,0.864723333035739,1.81316452000092E-5));
#115566=DIRECTION('ref_axis',(0.749703650686959,0.43543233401829,0.498340364247198));
#115567=DIRECTION('center_axis',(-1.4081690688991E-16,0.,-1.));
#115568=DIRECTION('ref_axis',(-1.,0.,1.16261524579732E-16));
#115569=DIRECTION('center_axis',(0.404349235495135,-0.914604666187785,1.84940535722811E-5));
#115570=DIRECTION('ref_axis',(0.792949544396578,0.350555095114516,-0.498339387697293));
#115571=DIRECTION('center_axis',(-0.502260184874095,0.86471654682158,1.85257151301963E-5));
#115572=DIRECTION('ref_axis',(0.748187385817233,0.434586366991526,-0.501348506858335));
#115573=DIRECTION('center_axis',(-1.4081690688991E-16,0.,-1.));
#115574=DIRECTION('ref_axis',(-1.,0.,1.40816906889911E-16));
#115575=DIRECTION('center_axis',(-1.4081690688991E-16,0.,-1.));
#115576=DIRECTION('ref_axis',(-1.,0.,1.4081690688991E-16));
#115577=DIRECTION('',(-0.866025403784442,-0.499999999999995,1.21951018649011E-16));
#115578=DIRECTION('center_axis',(-1.4081690688991E-16,0.,-1.));
#115579=DIRECTION('ref_axis',(-1.,0.,1.4081690688991E-16));
#115580=DIRECTION('center_axis',(-1.4081690688991E-16,0.,-1.));
#115581=DIRECTION('ref_axis',(-1.,0.,1.4081690688991E-16));
#115582=DIRECTION('center_axis',(-1.4081690688991E-16,0.,-1.));
#115583=DIRECTION('ref_axis',(-1.,0.,1.4081690688991E-16));
#115584=DIRECTION('',(0.80901699437495,0.587785252292469,-1.13923270769253E-16));
#115585=DIRECTION('center_axis',(1.4081690688991E-16,0.,1.));
#115586=DIRECTION('ref_axis',(1.,0.,-1.4081690688991E-16));
#115587=DIRECTION('',(-0.433019586648882,-0.249998457755582,0.866022406579796));
#115588=DIRECTION('center_axis',(1.4081690688991E-16,0.,1.));
#115589=DIRECTION('ref_axis',(-1.,0.,1.40816906889911E-16));
#115590=DIRECTION('',(0.40450988855993,0.293899542971733,-0.866022406579783));
#115591=DIRECTION('center_axis',(-1.4081690688991E-16,0.,-1.));
#115592=DIRECTION('ref_axis',(-1.,0.,1.40816906889911E-16));
#115593=DIRECTION('center_axis',(-1.4081690688991E-16,0.,-1.));
#115594=DIRECTION('ref_axis',(-1.,0.,1.4081690688991E-16));
#115595=DIRECTION('',(-0.866025403784442,-0.499999999999995,1.21951018649011E-16));
#115596=DIRECTION('center_axis',(1.4081690688991E-16,0.,1.));
#115597=DIRECTION('ref_axis',(-1.,8.88178419700125E-16,1.4081690688991E-16));
#115598=DIRECTION('',(0.80901699437495,0.587785252292469,-1.13923270769253E-16));
#115599=DIRECTION('center_axis',(-1.4081690688991E-16,0.,-1.));
#115600=DIRECTION('ref_axis',(-1.,0.,1.4081690688991E-16));
#115601=DIRECTION('center_axis',(-1.4081690688991E-16,0.,-1.));
#115602=DIRECTION('ref_axis',(1.,0.,-1.4081690688991E-16));
#115603=DIRECTION('',(-0.433014711050233,-0.250006503598672,-0.866022521746663));
#115604=DIRECTION('center_axis',(-1.4081690688991E-16,0.,-1.));
#115605=DIRECTION('ref_axis',(-1.,0.,1.4081690688991E-16));
#115606=DIRECTION('center_axis',(-1.4081690688991E-16,0.,-1.));
#115607=DIRECTION('ref_axis',(-1.,0.,1.4081690688991E-16));
#115608=DIRECTION('center_axis',(-1.4081690688991E-16,0.,-1.));
#115609=DIRECTION('ref_axis',(-1.,0.,1.4081690688991E-16));
#115610=DIRECTION('',(0.4045152557187,0.293891816351548,0.866022521746648));
#115611=DIRECTION('center_axis',(-1.4081690688991E-16,0.,-1.));
#115612=DIRECTION('ref_axis',(-1.,0.,1.40816906889911E-16));
#115613=DIRECTION('',(-0.866025403784442,-0.499999999999995,1.21951018649011E-16));
#115614=DIRECTION('center_axis',(1.4081690688991E-16,0.,1.));
#115615=DIRECTION('ref_axis',(-1.,0.,1.4081690688991E-16));
#115616=DIRECTION('',(0.80901699437495,0.587785252292469,-1.13923270769253E-16));
#115617=DIRECTION('center_axis',(-1.4081690688991E-16,0.,-1.));
#115618=DIRECTION('ref_axis',(-1.,0.,1.17174841180864E-16));
#115619=DIRECTION('center_axis',(-0.500926582476549,0.865489779781664,7.86457205664354E-6));
#115620=DIRECTION('ref_axis',(-5.2072675490952E-6,6.07299293807615E-6,-0.999999999968002));
#115621=DIRECTION('center_axis',(0.586919060371506,-0.809645611678824,7.86457244280782E-6));
#115622=DIRECTION('ref_axis',(0.686618216541034,0.497730297112336,-0.529924500330448));
#115623=DIRECTION('center_axis',(-1.4081690688991E-16,0.,-1.));
#115624=DIRECTION('ref_axis',(-1.,0.,1.13676889660403E-16));
#115625=DIRECTION('center_axis',(-0.500887108752517,0.86551262508994,-9.77058817878717E-6));
#115626=DIRECTION('ref_axis',(0.757015822393057,0.438092662174431,-0.484769908302365));
#115627=DIRECTION('center_axis',(0.586955986039185,-0.809618842639736,-9.7705214324476E-6));
#115628=DIRECTION('ref_axis',(0.708129726178571,0.513384442288636,-0.484756336026925));
#115629=DIRECTION('center_axis',(-1.4081690688991E-16,0.,-1.));
#115630=DIRECTION('ref_axis',(-1.,0.,1.15974593313694E-16));
#115631=DIRECTION('center_axis',(0.497748107605451,-0.867321636444818,1.81624796098486E-5));
#115632=DIRECTION('ref_axis',(0.750441041148855,0.430681881041565,0.501349539844131));
#115633=DIRECTION('center_axis',(-0.589885332530219,0.807487024129154,1.8131645283277E-5));
#115634=DIRECTION('ref_axis',(0.700081622909386,0.511412360641763,0.498340364256578));
#115635=DIRECTION('center_axis',(-1.4081690688991E-16,0.,-1.));
#115636=DIRECTION('ref_axis',(-1.,0.,1.16261524579732E-16));
#115637=DIRECTION('center_axis',(0.497736388330941,-0.867328361919083,1.84940567397459E-5));
#115638=DIRECTION('ref_axis',(0.751962698443092,0.431520514949629,-0.498339387694561));
#115639=DIRECTION('center_axis',(-0.589896242832074,0.807479053814649,1.85257114861555E-5));
#115640=DIRECTION('ref_axis',(0.698662091932204,0.510412535075371,-0.501348506864087));
#115641=DIRECTION('center_axis',(-1.4081690688991E-16,0.,-1.));
#115642=DIRECTION('ref_axis',(-1.,0.,1.40816906889911E-16));
#115643=DIRECTION('center_axis',(-1.4081690688991E-16,0.,-1.));
#115644=DIRECTION('ref_axis',(-1.,0.,1.4081690688991E-16));
#115645=DIRECTION('',(-0.80901699437495,-0.587785252292469,1.13923270769253E-16));
#115646=DIRECTION('center_axis',(-1.4081690688991E-16,0.,-1.));
#115647=DIRECTION('ref_axis',(-1.,0.,1.4081690688991E-16));
#115648=DIRECTION('center_axis',(-1.4081690688991E-16,0.,-1.));
#115649=DIRECTION('ref_axis',(-1.,0.,1.4081690688991E-16));
#115650=DIRECTION('center_axis',(-1.4081690688991E-16,0.,-1.));
#115651=DIRECTION('ref_axis',(-1.,0.,1.4081690688991E-16));
#115652=DIRECTION('',(0.743144825477398,0.669130606358854,-1.04647355694969E-16));
#115653=DIRECTION('center_axis',(1.4081690688991E-16,0.,1.));
#115654=DIRECTION('ref_axis',(1.,0.,-1.4081690688991E-16));
#115655=DIRECTION('',(-0.404515505437168,-0.293891812003425,0.866022406579793));
#115656=DIRECTION('center_axis',(1.4081690688991E-16,0.,1.));
#115657=DIRECTION('ref_axis',(-1.,8.88178419700125E-16,1.40816906889911E-16));
#115658=DIRECTION('',(0.371573073483921,0.334572327551833,-0.866022406579796));
#115659=DIRECTION('center_axis',(-1.4081690688991E-16,0.,-1.));
#115660=DIRECTION('ref_axis',(-1.,0.,1.40816906889911E-16));
#115661=DIRECTION('center_axis',(-1.4081690688991E-16,0.,-1.));
#115662=DIRECTION('ref_axis',(-1.,0.,1.4081690688991E-16));
#115663=DIRECTION('',(-0.80901699437495,-0.587785252292469,1.13923270769253E-16));
#115664=DIRECTION('center_axis',(1.4081690688991E-16,0.,1.));
#115665=DIRECTION('ref_axis',(-1.,0.,1.4081690688991E-16));
#115666=DIRECTION('',(0.743144825477398,0.669130606358854,-1.04647355694969E-16));
#115667=DIRECTION('center_axis',(-1.4081690688991E-16,0.,-1.));
#115668=DIRECTION('ref_axis',(-1.,0.,1.4081690688991E-16));
#115669=DIRECTION('center_axis',(-1.4081690688991E-16,0.,-1.));
#115670=DIRECTION('ref_axis',(1.,0.,-1.4081690688991E-16));
#115671=DIRECTION('',(-0.40450981552795,-0.293899304131695,-0.866022521746663));
#115672=DIRECTION('center_axis',(-1.4081690688991E-16,0.,-1.));
#115673=DIRECTION('ref_axis',(-1.,0.,1.4081690688991E-16));
#115674=DIRECTION('center_axis',(-1.4081690688991E-16,0.,-1.));
#115675=DIRECTION('ref_axis',(-1.,0.,1.4081690688991E-16));
#115676=DIRECTION('center_axis',(-1.4081690688991E-16,0.,-1.));
#115677=DIRECTION('ref_axis',(-1.,0.,1.4081690688991E-16));
#115678=DIRECTION('',(0.371579218892551,0.33456520427975,0.866022521746664));
#115679=DIRECTION('center_axis',(-1.4081690688991E-16,0.,-1.));
#115680=DIRECTION('ref_axis',(-1.,0.,1.40816906889911E-16));
#115681=DIRECTION('',(-0.80901699437495,-0.587785252292469,1.13923270769253E-16));
#115682=DIRECTION('center_axis',(1.4081690688991E-16,0.,1.));
#115683=DIRECTION('ref_axis',(-1.,0.,1.4081690688991E-16));
#115684=DIRECTION('',(0.743144825477398,0.669130606358854,-1.04647355694969E-16));
#115685=DIRECTION('center_axis',(-1.4081690688991E-16,0.,-1.));
#115686=DIRECTION('ref_axis',(-1.,0.,1.17174841180864E-16));
#115687=DIRECTION('center_axis',(-0.588650770899332,0.808387450334164,7.86457198365576E-6));
#115688=DIRECTION('ref_axis',(-5.81354222511576E-6,5.49541667256838E-6,
-0.999999999968002));
#115689=DIRECTION('center_axis',(0.66833486792867,-0.743860540860258,7.86457232182708E-6));
#115690=DIRECTION('ref_axis',(0.630829867029784,0.566774825493066,-0.529924500330461));
#115691=DIRECTION('center_axis',(-1.4081690688991E-16,0.,-1.));
#115692=DIRECTION('ref_axis',(-1.,0.,1.13676889660403E-16));
#115693=DIRECTION('center_axis',(-0.588613901404025,0.808414296619294,-9.77059377784101E-6));
#115694=DIRECTION('ref_axis',(0.707075657763069,0.514822445315911,-0.484769908304826));
#115695=DIRECTION('center_axis',(0.668368793190144,-0.743830058678787,-9.77051413964613E-6));
#115696=DIRECTION('ref_axis',(0.650587230627881,0.584591780669203,-0.484756336026621));
#115697=DIRECTION('center_axis',(-1.4081690688991E-16,0.,-1.));
#115698=DIRECTION('ref_axis',(-1.,0.,1.15974593313694E-16));
#115699=DIRECTION('center_axis',(0.585681189207983,-0.810541512988722,1.81624798474342E-5));
#115700=DIRECTION('ref_axis',(0.701311531424911,0.506765009439859,0.501349539840086));
#115701=DIRECTION('center_axis',(-0.671059256698738,0.741403718408655,1.81316454615391E-5));
#115702=DIRECTION('ref_axis',(0.642789354376861,0.581789246427063,0.498340364250789));
#115703=DIRECTION('center_axis',(-1.4081690688991E-16,0.,-1.));
#115704=DIRECTION('ref_axis',(-1.,0.,1.16261524579732E-16));
#115705=DIRECTION('center_axis',(0.585670237128126,-0.810549426623852,1.84940388037811E-5));
#115706=DIRECTION('ref_axis',(0.702737191804828,0.507758105720191,-0.498339387696485));
#115707=DIRECTION('center_axis',(-0.671069274112383,0.741394651315396,1.85257013794949E-5));
#115708=DIRECTION('ref_axis',(0.641482109968578,0.580646516617888,-0.501348506859026));
#115709=DIRECTION('center_axis',(-1.4081690688991E-16,0.,-1.));
#115710=DIRECTION('ref_axis',(-1.,0.,1.40816906889911E-16));
#115711=DIRECTION('center_axis',(-1.4081690688991E-16,0.,-1.));
#115712=DIRECTION('ref_axis',(-1.,0.,1.4081690688991E-16));
#115713=DIRECTION('',(-0.743144825477398,-0.669130606358854,1.04647355694969E-16));
#115714=DIRECTION('center_axis',(-1.4081690688991E-16,0.,-1.));
#115715=DIRECTION('ref_axis',(-1.,0.,1.4081690688991E-16));
#115716=DIRECTION('center_axis',(-1.4081690688991E-16,0.,-1.));
#115717=DIRECTION('ref_axis',(-1.,0.,1.4081690688991E-16));
#115718=DIRECTION('center_axis',(-1.4081690688991E-16,0.,-1.));
#115719=DIRECTION('ref_axis',(-1.,0.,1.4081690688991E-16));
#115720=DIRECTION('',(0.669130606358862,0.743144825477391,-9.42249022928252E-17));
#115721=DIRECTION('center_axis',(1.4081690688991E-16,0.,1.));
#115722=DIRECTION('ref_axis',(1.,0.,-1.4081690688991E-16));
#115723=DIRECTION('',(-0.371579467697564,-0.334565226058147,0.866022406579793));
#115724=DIRECTION('center_axis',(1.4081690688991E-16,0.,1.));
#115725=DIRECTION('ref_axis',(-1.,-8.88178419700125E-16,1.40816906889911E-16));
#115726=DIRECTION('',(0.334565226058151,0.371579467697541,-0.866022406579802));
#115727=DIRECTION('center_axis',(-1.4081690688991E-16,0.,-1.));
#115728=DIRECTION('ref_axis',(-1.,0.,1.40816906889911E-16));
#115729=DIRECTION('center_axis',(-1.4081690688991E-16,0.,-1.));
#115730=DIRECTION('ref_axis',(-1.,0.,1.4081690688991E-16));
#115731=DIRECTION('',(-0.743144825477398,-0.669130606358854,1.04647355694969E-16));
#115732=DIRECTION('center_axis',(1.4081690688991E-16,0.,1.));
#115733=DIRECTION('ref_axis',(-1.,0.,1.4081690688991E-16));
#115734=DIRECTION('',(0.669130606358862,0.743144825477391,-9.42249022928252E-17));
#115735=DIRECTION('center_axis',(-1.4081690688991E-16,0.,-1.));
#115736=DIRECTION('ref_axis',(-1.,0.,1.4081690688991E-16));
#115737=DIRECTION('center_axis',(-1.4081690688991E-16,0.,-1.));
#115738=DIRECTION('ref_axis',(1.,0.,-1.4081690688991E-16));
#115739=DIRECTION('',(-0.371573025817597,-0.334572082386321,-0.866022521746655));
#115740=DIRECTION('center_axis',(-1.4081690688991E-16,0.,-1.));
#115741=DIRECTION('ref_axis',(-1.,0.,1.4081690688991E-16));
#115742=DIRECTION('center_axis',(-1.4081690688991E-16,0.,-1.));
#115743=DIRECTION('ref_axis',(-1.,0.,1.4081690688991E-16));
#115744=DIRECTION('center_axis',(-1.4081690688991E-16,0.,-1.));
#115745=DIRECTION('ref_axis',(-1.,0.,1.4081690688991E-16));
#115746=DIRECTION('',(0.334572082386318,0.371573025817621,0.866022521746647));
#115747=DIRECTION('center_axis',(-1.4081690688991E-16,0.,-1.));
#115748=DIRECTION('ref_axis',(-1.,0.,1.40816906889911E-16));
#115749=DIRECTION('',(-0.743144825477398,-0.669130606358854,1.04647355694969E-16));
#115750=DIRECTION('center_axis',(1.4081690688991E-16,0.,1.));
#115751=DIRECTION('ref_axis',(-1.,-8.88178419700125E-16,1.4081690688991E-16));
#115752=DIRECTION('',(0.669130606358862,0.743144825477391,-9.42249022928252E-17));
#115753=DIRECTION('center_axis',(-1.4081690688991E-16,0.,-1.));
#115754=DIRECTION('ref_axis',(-1.,0.,1.17174841180864E-16));
#115755=DIRECTION('center_axis',(-0.669925578293108,0.742428258814812,7.86457198741695E-6));
#115756=DIRECTION('ref_axis',(-6.35612244774292E-6,4.85763161650682E-6,
-0.999999999968002));
#115757=DIRECTION('center_axis',(0.742428258814674,-0.669925578293261,7.86457238264939E-6));
#115758=DIRECTION('ref_axis',(0.568130013485845,0.629609650280319,-0.529924500330442));
#115759=DIRECTION('center_axis',(-1.4081690688991E-16,0.,-1.));
#115760=DIRECTION('ref_axis',(-1.,0.,1.13676889660403E-16));
#115761=DIRECTION('center_axis',(-0.669891716969178,0.742458811948934,-9.77058294495678E-6));
#115762=DIRECTION('ref_axis',(0.649388624262771,0.585911726013647,-0.48476990830477));
#115763=DIRECTION('center_axis',(0.742458811969791,-0.669891716946062,-9.77052667155945E-6));
#115764=DIRECTION('ref_axis',(0.58591676523382,0.649394209166528,-0.484756336027614));
#115765=DIRECTION('center_axis',(-1.4081690688991E-16,0.,-1.));
#115766=DIRECTION('ref_axis',(-1.,0.,1.15974593313694E-16));
#115767=DIRECTION('center_axis',(0.667197425140001,-0.744880927099545,1.81624799140914E-5));
#115768=DIRECTION('ref_axis',(0.644498305802315,0.577295914346694,0.501349539838784));
#115769=DIRECTION('center_axis',(-0.744880915222515,0.667197438400742,1.81316451171186E-5));
#115770=DIRECTION('ref_axis',(0.578454551163314,0.645791927479989,0.498340364249305));
#115771=DIRECTION('center_axis',(-1.4081690688991E-16,0.,-1.));
#115772=DIRECTION('ref_axis',(-1.,0.,1.16261524579732E-16));
#115773=DIRECTION('center_axis',(0.667187360268925,-0.744889942176261,1.84940667004621E-5));
#115774=DIRECTION('ref_axis',(0.645812349437408,0.578432592430395,-0.498339387695161));
#115775=DIRECTION('center_axis',(-0.744889929984212,0.667187373880017,1.85257177346086E-5));
#115776=DIRECTION('ref_axis',(0.577273915765294,0.644518813412645,-0.501348506863399));
#115777=DIRECTION('center_axis',(-1.4081690688991E-16,0.,-1.));
#115778=DIRECTION('ref_axis',(-1.,0.,1.40816906889911E-16));
#115779=DIRECTION('center_axis',(-1.4081690688991E-16,0.,-1.));
#115780=DIRECTION('ref_axis',(-1.,0.,1.4081690688991E-16));
#115781=DIRECTION('',(-0.669130606358862,-0.743144825477391,9.42249022928252E-17));
#115782=DIRECTION('center_axis',(-1.4081690688991E-16,0.,-1.));
#115783=DIRECTION('ref_axis',(-1.,0.,1.4081690688991E-16));
#115784=DIRECTION('center_axis',(-1.4081690688991E-16,0.,-1.));
#115785=DIRECTION('ref_axis',(-1.,0.,1.4081690688991E-16));
#115786=DIRECTION('center_axis',(-1.4081690688991E-16,0.,-1.));
#115787=DIRECTION('ref_axis',(-1.,0.,1.4081690688991E-16));
#115788=DIRECTION('',(0.587785252292477,0.809016994374945,-8.27701011433323E-17));
#115789=DIRECTION('center_axis',(1.4081690688991E-16,0.,1.));
#115790=DIRECTION('ref_axis',(1.,0.,-1.4081690688991E-16));
#115791=DIRECTION('',(-0.334572327551837,-0.371573073483898,0.866022406579805));
#115792=DIRECTION('center_axis',(1.4081690688991E-16,0.,1.));
#115793=DIRECTION('ref_axis',(-1.,-8.88178419700125E-16,1.40816906889911E-16));
#115794=DIRECTION('',(0.293891812003446,0.404515505437187,-0.866022406579777));
#115795=DIRECTION('center_axis',(-1.4081690688991E-16,0.,-1.));
#115796=DIRECTION('ref_axis',(-1.,0.,1.40816906889911E-16));
#115797=DIRECTION('center_axis',(-1.4081690688991E-16,0.,-1.));
#115798=DIRECTION('ref_axis',(-1.,0.,1.4081690688991E-16));
#115799=DIRECTION('',(-0.669130606358862,-0.743144825477391,9.42249022928252E-17));
#115800=DIRECTION('center_axis',(1.4081690688991E-16,0.,1.));
#115801=DIRECTION('ref_axis',(-1.,0.,1.4081690688991E-16));
#115802=DIRECTION('',(0.587785252292477,0.809016994374945,-8.27701011433323E-17));
#115803=DIRECTION('center_axis',(-1.4081690688991E-16,0.,-1.));
#115804=DIRECTION('ref_axis',(-1.,0.,1.4081690688991E-16));
#115805=DIRECTION('center_axis',(-1.4081690688991E-16,0.,-1.));
#115806=DIRECTION('ref_axis',(1.,0.,-1.4081690688991E-16));
#115807=DIRECTION('',(-0.334565204279747,-0.371579218892574,-0.866022521746655));
#115808=DIRECTION('center_axis',(-1.4081690688991E-16,0.,-1.));
#115809=DIRECTION('ref_axis',(-1.,0.,1.4081690688991E-16));
#115810=DIRECTION('center_axis',(-1.4081690688991E-16,0.,-1.));
#115811=DIRECTION('ref_axis',(-1.,0.,1.4081690688991E-16));
#115812=DIRECTION('center_axis',(-1.4081690688991E-16,0.,-1.));
#115813=DIRECTION('ref_axis',(-1.,0.,1.4081690688991E-16));
#115814=DIRECTION('',(0.293899304131692,0.404509815527973,0.866022521746654));
#115815=DIRECTION('center_axis',(-1.4081690688991E-16,0.,-1.));
#115816=DIRECTION('ref_axis',(-1.,0.,1.40816906889911E-16));
#115817=DIRECTION('',(-0.669130606358862,-0.743144825477391,9.42249022928252E-17));
#115818=DIRECTION('center_axis',(1.4081690688991E-16,0.,1.));
#115819=DIRECTION('ref_axis',(-1.,0.,1.4081690688991E-16));
#115820=DIRECTION('',(0.587785252292477,0.809016994374945,-8.27701011433323E-17));
#115821=DIRECTION('center_axis',(-1.4081690688991E-16,0.,-1.));
#115822=DIRECTION('ref_axis',(-1.,0.,1.17174841180864E-16));
#115823=DIRECTION('center_axis',(-0.743860540860165,0.668334867928774,7.86457206040205E-6));
#115824=DIRECTION('ref_axis',(-6.82906381692535E-6,4.16662528541507E-6,
-0.999999999968002));
#115825=DIRECTION('center_axis',(0.808387450334043,-0.588650770899498,7.86457228997828E-6));
#115826=DIRECTION('ref_axis',(0.499205608625192,0.685546339984894,-0.529924500330441));
#115827=DIRECTION('center_axis',(-1.4081690688991E-16,0.,-1.));
#115828=DIRECTION('ref_axis',(-1.,0.,1.13676889660403E-16));
#115829=DIRECTION('center_axis',(-0.743830058703291,0.668368793162873,-9.7705803850988E-6));
#115830=DIRECTION('ref_axis',(0.584586753102978,0.650581635232684,-0.484769908301335));
#115831=DIRECTION('center_axis',(0.80841429664589,-0.588613901367499,-9.77051216005777E-6));
#115832=DIRECTION('ref_axis',(0.514826873149602,0.707081738814493,-0.484756336026747));
#115833=DIRECTION('center_axis',(-1.4081690688991E-16,0.,-1.));
#115834=DIRECTION('ref_axis',(-1.,0.,1.15974593313694E-16));
#115835=DIRECTION('center_axis',(0.741403706462381,-0.671059269896459,1.8162479445365E-5));
#115836=DIRECTION('ref_axis',(0.580623821869585,0.641501844407272,0.501349539841839));
#115837=DIRECTION('center_axis',(-0.810541502562996,0.585681203637409,1.8131645405925E-5));
#115838=DIRECTION('ref_axis',(0.507782078838539,0.702719177036071,0.49834036424532));
#115839=DIRECTION('center_axis',(-1.4081690688991E-16,0.,-1.));
#115840=DIRECTION('ref_axis',(-1.,0.,1.16261524579732E-16));
#115841=DIRECTION('center_axis',(0.741394639062402,-0.671069287650314,1.84940740269212E-5));
#115842=DIRECTION('ref_axis',(0.581811851821584,0.642769650609807,-0.498339387701681));
#115843=DIRECTION('center_axis',(-0.810549415915106,0.585670251947697,1.85257082024649E-5));
#115844=DIRECTION('ref_axis',(0.506740987742068,0.701329627217269,-0.501348506858732));
#115845=DIRECTION('center_axis',(-1.4081690688991E-16,0.,-1.));
#115846=DIRECTION('ref_axis',(-1.,0.,1.40816906889911E-16));
#115847=DIRECTION('center_axis',(-1.4081690688991E-16,0.,-1.));
#115848=DIRECTION('ref_axis',(-1.,0.,1.4081690688991E-16));
#115849=DIRECTION('',(-0.587785252292477,-0.809016994374945,8.27701011433323E-17));
#115850=DIRECTION('center_axis',(-1.4081690688991E-16,0.,-1.));
#115851=DIRECTION('ref_axis',(-1.,0.,1.4081690688991E-16));
#115852=DIRECTION('center_axis',(-1.4081690688991E-16,0.,-1.));
#115853=DIRECTION('ref_axis',(-1.,0.,1.4081690688991E-16));
#115854=DIRECTION('center_axis',(-1.4081690688991E-16,0.,-1.));
#115855=DIRECTION('ref_axis',(-1.,0.,1.4081690688991E-16));
#115856=DIRECTION('',(0.500000000000004,0.866025403784436,-7.04084534449558E-17));
#115857=DIRECTION('center_axis',(1.4081690688991E-16,0.,1.));
#115858=DIRECTION('ref_axis',(1.,0.,-1.4081690688991E-16));
#115859=DIRECTION('',(-0.293899542971745,-0.404509888559929,0.86602240657978));
#115860=DIRECTION('center_axis',(1.4081690688991E-16,0.,1.));
#115861=DIRECTION('ref_axis',(-1.,0.,1.40816906889911E-16));
#115862=DIRECTION('',(0.249998457755608,0.433019586648879,-0.866022406579791));
#115863=DIRECTION('center_axis',(-1.4081690688991E-16,0.,-1.));
#115864=DIRECTION('ref_axis',(-1.,0.,1.40816906889911E-16));
#115865=DIRECTION('center_axis',(-1.4081690688991E-16,0.,-1.));
#115866=DIRECTION('ref_axis',(-1.,0.,1.4081690688991E-16));
#115867=DIRECTION('',(-0.587785252292477,-0.809016994374945,8.27701011433323E-17));
#115868=DIRECTION('center_axis',(1.4081690688991E-16,0.,1.));
#115869=DIRECTION('ref_axis',(-1.,1.77635683940025E-15,1.4081690688991E-16));
#115870=DIRECTION('',(0.500000000000004,0.866025403784436,-7.04084534449558E-17));
#115871=DIRECTION('center_axis',(-1.4081690688991E-16,0.,-1.));
#115872=DIRECTION('ref_axis',(-1.,0.,1.4081690688991E-16));
#115873=DIRECTION('center_axis',(-1.4081690688991E-16,0.,-1.));
#115874=DIRECTION('ref_axis',(1.,1.06581410364015E-14,-1.4081690688991E-16));
#115875=DIRECTION('',(-0.293891816351505,-0.404515255718661,-0.866022521746681));
#115876=DIRECTION('center_axis',(-1.4081690688991E-16,0.,-1.));
#115877=DIRECTION('ref_axis',(-1.,0.,1.4081690688991E-16));
#115878=DIRECTION('center_axis',(-1.4081690688991E-16,0.,-1.));
#115879=DIRECTION('ref_axis',(-1.,0.,1.4081690688991E-16));
#115880=DIRECTION('center_axis',(-1.4081690688991E-16,0.,-1.));
#115881=DIRECTION('ref_axis',(-1.,0.,1.4081690688991E-16));
#115882=DIRECTION('',(0.250006503598672,0.433014711050233,0.866022521746663));
#115883=DIRECTION('center_axis',(-1.4081690688991E-16,0.,-1.));
#115884=DIRECTION('ref_axis',(-1.,0.,1.40816906889911E-16));
#115885=DIRECTION('',(-0.587785252292477,-0.809016994374945,8.27701011433323E-17));
#115886=DIRECTION('center_axis',(1.4081690688991E-16,0.,1.));
#115887=DIRECTION('ref_axis',(-1.,0.,1.4081690688991E-16));
#115888=DIRECTION('',(0.500000000000004,0.866025403784436,-7.04084534449558E-17));
#115889=DIRECTION('center_axis',(-1.4081690688991E-16,0.,-1.));
#115890=DIRECTION('ref_axis',(-1.,0.,1.17174841180864E-16));
#115891=DIRECTION('center_axis',(-0.809645611678678,0.586919060371707,7.8645720234677E-6));
#115892=DIRECTION('ref_axis',(-7.22718435185782E-6,3.42996856068737E-6,
-0.999999999968002));
#115893=DIRECTION('center_axis',(0.865489779781566,-0.500926582476719,7.86457236031111E-6));
#115894=DIRECTION('ref_axis',(0.424811802651068,0.7339720405287,-0.529924500330459));
#115895=DIRECTION('center_axis',(-1.4081690688991E-16,0.,-1.));
#115896=DIRECTION('ref_axis',(-1.,0.,1.13676889660403E-16));
#115897=DIRECTION('center_axis',(-0.80961884266152,0.586955986009136,-9.77058844484673E-6));
#115898=DIRECTION('ref_axis',(0.513380027141697,0.708123635911376,-0.48476990830253));
#115899=DIRECTION('center_axis',(0.865512625110006,-0.500887108717845,-9.77051580085054E-6));
#115900=DIRECTION('ref_axis',(0.438096430108505,0.757022332965597,-0.484756336026162));
#115901=DIRECTION('center_axis',(-1.4081690688991E-16,0.,-1.));
#115902=DIRECTION('ref_axis',(-1.,0.,1.15974593313694E-16));
#115903=DIRECTION('center_axis',(0.807487013627689,-0.5898853469046,1.81624798587448E-5));
#115904=DIRECTION('ref_axis',(0.510387901843966,0.698679346020879,0.501349539837378));
#115905=DIRECTION('center_axis',(-0.867321627584491,0.497748123045615,1.81316450671902E-5));
#115906=DIRECTION('ref_axis',(0.43154623979482,0.751947288230966,0.498340364250227));
#115907=DIRECTION('center_axis',(-1.4081690688991E-16,0.,-1.));
#115908=DIRECTION('ref_axis',(-1.,0.,1.16261524579732E-16));
#115909=DIRECTION('center_axis',(0.807479043031469,-0.589896257593616,1.84940475522698E-5));
#115910=DIRECTION('ref_axis',(0.511436901808568,0.700064389992322,-0.498339387699921));
#115911=DIRECTION('center_axis',(-0.867328352820218,0.497736404184951,1.85257186195537E-5));
#115912=DIRECTION('ref_axis',(0.430656099410934,0.750456526858012,-0.501348506865604));
#115913=DIRECTION('center_axis',(-1.4081690688991E-16,0.,-1.));
#115914=DIRECTION('ref_axis',(-1.,0.,1.40816906889911E-16));
#115915=DIRECTION('center_axis',(-1.4081690688991E-16,0.,-1.));
#115916=DIRECTION('ref_axis',(-1.,0.,1.4081690688991E-16));
#115917=DIRECTION('',(-0.500000000000004,-0.866025403784436,7.04084534449558E-17));
#115918=DIRECTION('center_axis',(-1.4081690688991E-16,0.,-1.));
#115919=DIRECTION('ref_axis',(-1.,0.,1.4081690688991E-16));
#115920=DIRECTION('center_axis',(-1.4081690688991E-16,0.,-1.));
#115921=DIRECTION('ref_axis',(-1.,0.,1.4081690688991E-16));
#115922=DIRECTION('center_axis',(-1.4081690688991E-16,0.,-1.));
#115923=DIRECTION('ref_axis',(-1.,0.,1.4081690688991E-16));
#115924=DIRECTION('',(0.406736643075804,0.913545457642599,-5.72753959967203E-17));
#115925=DIRECTION('center_axis',(1.4081690688991E-16,0.,1.));
#115926=DIRECTION('ref_axis',(1.,0.,-1.4081690688991E-16));
#115927=DIRECTION('',(-0.250006733496389,-0.433014808647754,0.866022406579769));
#115928=DIRECTION('center_axis',(1.4081690688991E-16,0.,1.));
#115929=DIRECTION('ref_axis',(-1.,0.,1.40816906889911E-16));
#115930=DIRECTION('',(0.203366068089046,0.45677941465413,-0.866022406579779));
#115931=DIRECTION('center_axis',(-1.4081690688991E-16,0.,-1.));
#115932=DIRECTION('ref_axis',(-1.,0.,1.40816906889911E-16));
#115933=DIRECTION('center_axis',(-1.4081690688991E-16,0.,-1.));
#115934=DIRECTION('ref_axis',(-1.,0.,1.4081690688991E-16));
#115935=DIRECTION('',(-0.500000000000004,-0.866025403784436,7.04084534449558E-17));
#115936=DIRECTION('center_axis',(1.4081690688991E-16,0.,1.));
#115937=DIRECTION('ref_axis',(-1.,0.,1.4081690688991E-16));
#115938=DIRECTION('',(0.406736643075804,0.913545457642599,-5.72753959967203E-17));
#115939=DIRECTION('center_axis',(-1.4081690688991E-16,0.,-1.));
#115940=DIRECTION('ref_axis',(-1.,0.,1.4081690688991E-16));
#115941=DIRECTION('center_axis',(-1.4081690688991E-16,0.,-1.));
#115942=DIRECTION('ref_axis',(1.,-4.44089209850063E-15,-1.4081690688991E-16));
#115943=DIRECTION('',(-0.249998488182553,-0.433019338752928,-0.866022521746643));
#115944=DIRECTION('center_axis',(-1.4081690688991E-16,0.,-1.));
#115945=DIRECTION('ref_axis',(-1.,0.,1.4081690688991E-16));
#115946=DIRECTION('center_axis',(-1.4081690688991E-16,0.,-1.));
#115947=DIRECTION('ref_axis',(-1.,0.,1.4081690688991E-16));
#115948=DIRECTION('center_axis',(-1.4081690688991E-16,0.,-1.));
#115949=DIRECTION('ref_axis',(-1.,0.,1.4081690688991E-16));
#115950=DIRECTION('',(0.203374579494966,0.456775406784138,0.866022521746653));
#115951=DIRECTION('center_axis',(-1.4081690688991E-16,0.,-1.));
#115952=DIRECTION('ref_axis',(-1.,0.,1.40816906889911E-16));
#115953=DIRECTION('',(-0.500000000000004,-0.866025403784436,7.04084534449558E-17));
#115954=DIRECTION('center_axis',(1.4081690688991E-16,0.,1.));
#115955=DIRECTION('ref_axis',(-1.,0.,1.4081690688991E-16));
#115956=DIRECTION('',(0.406736643075804,0.913545457642599,-5.72753959967203E-17));
#115957=DIRECTION('center_axis',(-1.4081690688991E-16,0.,-1.));
#115958=DIRECTION('ref_axis',(-1.,0.,1.17174841180864E-16));
#115959=DIRECTION('center_axis',(-0.866560035746417,0.499072844768494,7.864571930576E-6));
#115960=DIRECTION('ref_axis',(-7.54612234082935E-6,2.65573232063934E-6,
-0.999999999968002));
#115961=DIRECTION('center_axis',(0.913109622086463,-0.407714137590624,7.86457226365977E-6));
#115962=DIRECTION('ref_axis',(0.345763669669371,0.774356189803027,-0.52992450033048));
#115963=DIRECTION('center_axis',(-1.4081690688991E-16,0.,-1.));
#115964=DIRECTION('ref_axis',(-1.,0.,1.13676889660403E-16));
#115965=DIRECTION('center_axis',(-0.866537273152129,0.499112366248933,-9.77058580781023E-6));
#115966=DIRECTION('ref_axis',(0.43654860217199,0.757907285851209,-0.484769908302212));
#115967=DIRECTION('center_axis',(0.913128216134706,-0.407672492085481,-9.77051458842593E-6));
#115968=DIRECTION('ref_axis',(0.35656611090134,0.798668832019239,-0.484756336026378));
#115969=DIRECTION('center_axis',(-1.4081690688991E-16,0.,-1.));
#115970=DIRECTION('ref_axis',(-1.,0.,1.15974593313694E-16));
#115971=DIRECTION('center_axis',(0.864723324094319,-0.502248516610449,1.81624797599045E-5));
#115972=DIRECTION('ref_axis',(0.434560065156467,0.748201970505921,0.501349539844472));
#115973=DIRECTION('center_axis',(-0.914599195355502,0.404361609857206,1.81316449875146E-5));
#115974=DIRECTION('ref_axis',(0.350582289842569,0.792936907582701,0.498340364251104));
#115975=DIRECTION('center_axis',(-1.4081690688991E-16,0.,-1.));
#115976=DIRECTION('ref_axis',(-1.,0.,1.16261524579732E-16));
#115977=DIRECTION('center_axis',(0.864716537645395,-0.502260200673446,1.84940682125922E-5));
#115978=DIRECTION('ref_axis',(0.435458542073553,0.749689077419333,-0.498339387700114));
#115979=DIRECTION('center_axis',(-0.914604658797229,0.404349252210514,1.85257100784132E-5));
#115980=DIRECTION('ref_axis',(0.349852852737583,0.791361267753224,-0.501348506860632));
#115981=DIRECTION('center_axis',(-1.4081690688991E-16,0.,-1.));
#115982=DIRECTION('ref_axis',(-1.,0.,1.40816906889911E-16));
#115983=DIRECTION('center_axis',(-1.4081690688991E-16,0.,-1.));
#115984=DIRECTION('ref_axis',(-1.,0.,1.4081690688991E-16));
#115985=DIRECTION('',(-0.406736643075804,-0.913545457642599,5.72753959967203E-17));
#115986=DIRECTION('center_axis',(-1.4081690688991E-16,0.,-1.));
#115987=DIRECTION('ref_axis',(-1.,0.,1.4081690688991E-16));
#115988=DIRECTION('center_axis',(-1.4081690688991E-16,0.,-1.));
#115989=DIRECTION('ref_axis',(-1.,0.,1.4081690688991E-16));
#115990=DIRECTION('center_axis',(-1.4081690688991E-16,0.,-1.));
#115991=DIRECTION('ref_axis',(-1.,0.,1.4081690688991E-16));
#115992=DIRECTION('',(0.309016994374951,0.951056516295152,-4.35148173242975E-17));
#115993=DIRECTION('center_axis',(1.4081690688991E-16,0.,1.));
#115994=DIRECTION('ref_axis',(1.,0.,-1.4081690688991E-16));
#115995=DIRECTION('',(-0.203374797931583,-0.456775527877804,0.866022406579785));
#115996=DIRECTION('center_axis',(1.4081690688991E-16,0.,1.));
#115997=DIRECTION('ref_axis',(-1.,0.,1.40816906889911E-16));
#115998=DIRECTION('',(0.154505557223423,0.475534671805167,-0.866022406579779));
#115999=DIRECTION('center_axis',(-1.4081690688991E-16,0.,-1.));
#116000=DIRECTION('ref_axis',(-1.,0.,1.40816906889911E-16));
#116001=DIRECTION('center_axis',(-1.4081690688991E-16,0.,-1.));
#116002=DIRECTION('ref_axis',(-1.,0.,1.4081690688991E-16));
#116003=DIRECTION('',(-0.406736643075804,-0.913545457642599,5.72753959967203E-17));
#116004=DIRECTION('center_axis',(1.4081690688991E-16,0.,1.));
#116005=DIRECTION('ref_axis',(-1.,0.,1.4081690688991E-16));
#116006=DIRECTION('',(0.309016994374951,0.951056516295152,-4.35148173242975E-17));
#116007=DIRECTION('center_axis',(-1.4081690688991E-16,0.,-1.));
#116008=DIRECTION('ref_axis',(-1.,0.,1.4081690688991E-16));
#116009=DIRECTION('center_axis',(-1.4081690688991E-16,0.,-1.));
#116010=DIRECTION('ref_axis',(1.,0.,-1.4081690688991E-16));
#116011=DIRECTION('',(-0.203366124261498,-0.456779171296627,-0.866022521746648));
#116012=DIRECTION('center_axis',(-1.4081690688991E-16,0.,-1.));
#116013=DIRECTION('ref_axis',(-1.,0.,1.4081690688991E-16));
#116014=DIRECTION('center_axis',(-1.4081690688991E-16,0.,-1.));
#116015=DIRECTION('ref_axis',(-1.,0.,1.4081690688991E-16));
#116016=DIRECTION('center_axis',(-1.4081690688991E-16,0.,-1.));
#116017=DIRECTION('ref_axis',(-1.,0.,1.4081690688991E-16));
#116018=DIRECTION('',(0.15451444093947,0.475531575574902,0.866022521746643));
#116019=DIRECTION('center_axis',(-1.4081690688991E-16,0.,-1.));
#116020=DIRECTION('ref_axis',(-1.,0.,1.40816906889911E-16));
#116021=DIRECTION('',(-0.406736643075804,-0.913545457642599,5.72753959967203E-17));
#116022=DIRECTION('center_axis',(1.4081690688991E-16,0.,1.));
#116023=DIRECTION('ref_axis',(-1.,0.,1.4081690688991E-16));
#116024=DIRECTION('',(0.309016994374951,0.951056516295152,-4.35148173242975E-17));
#116025=DIRECTION('center_axis',(-1.4081690688991E-16,0.,-1.));
#116026=DIRECTION('ref_axis',(-1.,0.,1.17174841180864E-16));
#116027=DIRECTION('center_axis',(-0.913980246723224,0.405758682640191,7.86457205741761E-6));
#116028=DIRECTION('ref_axis',(-7.78238362395477E-6,1.85239942789989E-6,
-0.999999999968002));
#116029=DIRECTION('center_axis',(0.950725244291261,-0.310034691293524,7.86457240211258E-6));
#116030=DIRECTION('ref_axis',(0.262927277567292,0.806256330617353,-0.529924500330466));
#116031=DIRECTION('center_axis',(-1.4081690688991E-16,0.,-1.));
#116032=DIRECTION('ref_axis',(-1.,0.,1.13676889660403E-16));
#116033=DIRECTION('center_axis',(-0.913961739944989,0.405800366955557,-9.77058836349E-6));
#116034=DIRECTION('ref_axis',(0.354934259362683,0.79938714496408,-0.484769908303766));
#116035=DIRECTION('center_axis',(0.950739383338138,-0.309991330321275,-9.77051800065362E-6));
#116036=DIRECTION('ref_axis',(0.271129178766871,0.831564948216897,-0.484756336026907));
#116037=DIRECTION('center_axis',(-1.4081690688991E-16,0.,-1.));
#116038=DIRECTION('ref_axis',(-1.,0.,1.15974593313694E-16));
#116039=DIRECTION('center_axis',(0.912485544867189,-0.40910894646604,1.81624796870615E-5));
#116040=DIRECTION('ref_axis',(0.353971097459556,0.789527137633167,0.501349539846259));
#116041=DIRECTION('center_axis',(-0.951856222950115,0.306544826252842,1.81316453251061E-5));
#116042=DIRECTION('ref_axis',(0.265777286959374,0.825238944243956,0.498340364248808));
#116043=DIRECTION('center_axis',(-1.4081690688991E-16,0.,-1.));
#116044=DIRECTION('ref_axis',(-1.,0.,1.16261524579732E-16));
#116045=DIRECTION('center_axis',(0.912480016913587,-0.409121275896707,1.84940738513807E-5));
#116046=DIRECTION('ref_axis',(0.354709207426179,0.791100014431713,-0.498339387700025));
#116047=DIRECTION('center_axis',(-0.951860364736054,0.306531965219525,1.85257135621031E-5));
#116048=DIRECTION('ref_axis',(0.265216544996839,0.823595688993674,-0.501348506860223));
#116049=DIRECTION('center_axis',(-1.4081690688991E-16,0.,-1.));
#116050=DIRECTION('ref_axis',(-1.,0.,1.40816906889911E-16));
#116051=DIRECTION('center_axis',(-1.4081690688991E-16,0.,-1.));
#116052=DIRECTION('ref_axis',(-1.,0.,1.4081690688991E-16));
#116053=DIRECTION('',(-0.309016994374951,-0.951056516295152,4.35148173242975E-17));
#116054=DIRECTION('center_axis',(-1.4081690688991E-16,0.,-1.));
#116055=DIRECTION('ref_axis',(-1.,0.,1.4081690688991E-16));
#116056=DIRECTION('center_axis',(-1.4081690688991E-16,0.,-1.));
#116057=DIRECTION('ref_axis',(-1.,0.,1.4081690688991E-16));
#116058=DIRECTION('center_axis',(-1.4081690688991E-16,0.,-1.));
#116059=DIRECTION('ref_axis',(-1.,0.,1.4081690688991E-16));
#116060=DIRECTION('',(0.207911690817763,0.978147600733805,-2.92774812072088E-17));
#116061=DIRECTION('center_axis',(1.4081690688991E-16,0.,1.));
#116062=DIRECTION('ref_axis',(1.,0.,-1.4081690688991E-16));
#116063=DIRECTION('',(-0.154514645521709,-0.475531718838051,0.866022406579778));
#116064=DIRECTION('center_axis',(1.4081690688991E-16,0.,1.));
#116065=DIRECTION('ref_axis',(-1.,0.,1.40816906889911E-16));
#116066=DIRECTION('',(0.103952251140481,0.489079871579878,-0.866022406579781));
#116067=DIRECTION('center_axis',(-1.4081690688991E-16,0.,-1.));
#116068=DIRECTION('ref_axis',(-1.,0.,1.40816906889911E-16));
#116069=DIRECTION('center_axis',(-1.4081690688991E-16,0.,-1.));
#116070=DIRECTION('ref_axis',(-1.,0.,1.4081690688991E-16));
#116071=DIRECTION('',(-0.309016994374951,-0.951056516295152,4.35148173242975E-17));
#116072=DIRECTION('center_axis',(1.4081690688991E-16,0.,1.));
#116073=DIRECTION('ref_axis',(-1.,0.,1.4081690688991E-16));
#116074=DIRECTION('',(0.207911690817763,0.978147600733805,-2.92774812072088E-17));
#116075=DIRECTION('center_axis',(-1.4081690688991E-16,0.,-1.));
#116076=DIRECTION('ref_axis',(-1.,0.,1.4081690688991E-16));
#116077=DIRECTION('center_axis',(-1.4081690688991E-16,0.,-1.));
#116078=DIRECTION('ref_axis',(1.,0.,-1.4081690688991E-16));
#116079=DIRECTION('',(-0.154505638525953,-0.47553443565238,-0.866022521746669));
#116080=DIRECTION('center_axis',(-1.4081690688991E-16,0.,-1.));
#116081=DIRECTION('ref_axis',(-1.,0.,1.4081690688991E-16));
#116082=DIRECTION('center_axis',(-1.4081690688991E-16,0.,-1.));
#116083=DIRECTION('ref_axis',(-1.,0.,1.4081690688991E-16));
#116084=DIRECTION('center_axis',(-1.4081690688991E-16,0.,-1.));
#116085=DIRECTION('ref_axis',(-1.,0.,1.4081690688991E-16));
#116086=DIRECTION('',(0.103961409834823,0.489077720912261,0.866022521746648));
#116087=DIRECTION('center_axis',(-1.4081690688991E-16,0.,-1.));
#116088=DIRECTION('ref_axis',(-1.,0.,1.40816906889911E-16));
#116089=DIRECTION('',(-0.309016994374951,-0.951056516295152,4.35148173242975E-17));
#116090=DIRECTION('center_axis',(1.4081690688991E-16,0.,1.));
#116091=DIRECTION('ref_axis',(-1.,0.,1.4081690688991E-16));
#116092=DIRECTION('',(0.207911690817763,0.978147600733805,-2.92774812072088E-17));
#116093=DIRECTION('center_axis',(-1.4081690688991E-16,0.,-1.));
#116094=DIRECTION('ref_axis',(-1.,0.,1.17174841180864E-16));
#116095=DIRECTION('center_axis',(-0.951386698854225,0.307998943474501,7.864572011635E-6));
#116096=DIRECTION('ref_axis',(-7.93337934383608E-6,1.02877115701162E-6,
-0.999999999968002));
#116097=DIRECTION('center_axis',(0.977924521767603,-0.208958440039532,7.86457222572879E-6));
#116098=DIRECTION('ref_axis',(0.177210199190827,0.829322958353529,-0.529924500330471));
#116099=DIRECTION('center_axis',(-1.4081690688991E-16,0.,-1.));
#116100=DIRECTION('ref_axis',(-1.,0.,1.13676889660403E-16));
#116101=DIRECTION('center_axis',(-0.951372650655541,0.308042333923741,-9.77058865395253E-6));
#116102=DIRECTION('ref_axis',(0.269431182533353,0.832108751234505,-0.48476990830458));
#116103=DIRECTION('center_axis',(0.977934050903516,-0.20891383867034,-9.77051776669988E-6));
#116104=DIRECTION('ref_axis',(0.182721698612496,0.855350264825962,-0.484756336026998));
#116105=DIRECTION('center_axis',(-1.4081690688991E-16,0.,-1.));
#116106=DIRECTION('ref_axis',(-1.,0.,1.15974593313694E-16));
#116107=DIRECTION('center_axis',(0.950250383060633,-0.311487093092547,1.8162479704961E-5));
#116108=DIRECTION('ref_axis',(0.269503948348138,0.822202080228475,0.501349539834967));
#116109=DIRECTION('center_axis',(-0.978684514577286,0.205369473383621,1.81316451935691E-5));
#116110=DIRECTION('ref_axis',(0.178060372501543,0.848499490335405,0.498340364254362));
#116111=DIRECTION('center_axis',(-1.4081690688991E-16,0.,-1.));
#116112=DIRECTION('ref_axis',(-1.,0.,1.16261524579732E-16));
#116113=DIRECTION('center_axis',(0.950246174164968,-0.311499932813493,1.84940671105159E-5));
#116114=DIRECTION('ref_axis',(0.270073604475392,0.823843494140517,-0.498339387694785));
#116115=DIRECTION('center_axis',(-0.978687289329486,0.205356249872508,1.85257182595835E-5));
#116116=DIRECTION('ref_axis',(0.177674469289135,0.846806623517853,-0.50134850685837));
#116117=DIRECTION('center_axis',(-1.4081690688991E-16,0.,-1.));
#116118=DIRECTION('ref_axis',(-1.,0.,1.40816906889911E-16));
#116119=DIRECTION('center_axis',(-1.4081690688991E-16,0.,-1.));
#116120=DIRECTION('ref_axis',(-1.,0.,1.4081690688991E-16));
#116121=DIRECTION('',(-0.207911690817763,-0.978147600733805,2.92774812072088E-17));
#116122=DIRECTION('center_axis',(-1.4081690688991E-16,0.,-1.));
#116123=DIRECTION('ref_axis',(-1.,0.,1.4081690688991E-16));
#116124=DIRECTION('center_axis',(-1.4081690688991E-16,0.,-1.));
#116125=DIRECTION('ref_axis',(-1.,0.,1.4081690688991E-16));
#116126=DIRECTION('center_axis',(-1.4081690688991E-16,0.,-1.));
#116127=DIRECTION('ref_axis',(-1.,0.,1.4081690688991E-16));
#116128=DIRECTION('',(0.104528463267657,0.994521895368273,-1.47193748793071E-17));
#116129=DIRECTION('center_axis',(1.4081690688991E-16,0.,1.));
#116130=DIRECTION('ref_axis',(1.,0.,-1.4081690688991E-16));
#116131=DIRECTION('',(-0.103961598321241,-0.489077884775271,0.866022406579783));
#116132=DIRECTION('center_axis',(1.4081690688991E-16,0.,1.));
#116133=DIRECTION('ref_axis',(-1.,0.,1.40816906889911E-16));
#116134=DIRECTION('',(0.0522600224406464,0.497266609935041,-0.866022406579769));
#116135=DIRECTION('center_axis',(-1.4081690688991E-16,0.,-1.));
#116136=DIRECTION('ref_axis',(-1.,0.,1.40816906889911E-16));
#116137=DIRECTION('center_axis',(-1.4081690688991E-16,0.,-1.));
#116138=DIRECTION('ref_axis',(-1.,0.,1.4081690688991E-16));
#116139=DIRECTION('',(-0.207911690817763,-0.978147600733805,2.92774812072088E-17));
#116140=DIRECTION('center_axis',(1.4081690688991E-16,0.,1.));
#116141=DIRECTION('ref_axis',(-1.,0.,1.4081690688991E-16));
#116142=DIRECTION('',(0.104528463267657,0.994521895368273,-1.47193748793071E-17));
#116143=DIRECTION('center_axis',(-1.4081690688991E-16,0.,-1.));
#116144=DIRECTION('ref_axis',(-1.,0.,1.4081690688991E-16));
#116145=DIRECTION('center_axis',(-1.4081690688991E-16,0.,-1.));
#116146=DIRECTION('ref_axis',(1.,0.,-1.4081690688991E-16));
#116147=DIRECTION('',(-0.103952356682307,-0.489079645219225,-0.866022521746653));
#116148=DIRECTION('center_axis',(-1.4081690688991E-16,0.,-1.));
#116149=DIRECTION('ref_axis',(-1.,0.,1.4081690688991E-16));
#116150=DIRECTION('center_axis',(-1.4081690688991E-16,0.,-1.));
#116151=DIRECTION('ref_axis',(-1.,0.,1.4081690688991E-16));
#116152=DIRECTION('center_axis',(-1.4081690688991E-16,0.,-1.));
#116153=DIRECTION('ref_axis',(-1.,0.,1.4081690688991E-16));
#116154=DIRECTION('',(0.0522693557686676,0.497265428393217,0.866022521746657));
#116155=DIRECTION('center_axis',(-1.4081690688991E-16,0.,-1.));
#116156=DIRECTION('ref_axis',(-1.,0.,1.40816906889911E-16));
#116157=DIRECTION('',(-0.207911690817763,-0.978147600733805,2.92774812072088E-17));
#116158=DIRECTION('center_axis',(1.4081690688991E-16,0.,1.));
#116159=DIRECTION('ref_axis',(-1.,0.,1.4081690688991E-16));
#116160=DIRECTION('',(0.104528463267657,0.994521895368273,-1.47193748793071E-17));
#116161=DIRECTION('center_axis',(-1.4081690688991E-16,0.,-1.));
#116162=DIRECTION('ref_axis',(-1.,0.,1.17174841180864E-16));
#116163=DIRECTION('center_axis',(-0.978369559222116,0.206864703431182,7.86457201672164E-6));
#116164=DIRECTION('ref_axis',(-7.99745533554544E-6,1.93871482032992E-7,
-0.999999999968002));
#116165=DIRECTION('center_axis',(0.994409453539565,-0.105592796389204,7.86457224839845E-6));
#116166=DIRECTION('ref_axis',(0.0895515687885955,0.843303350210959,-0.529924500330448));
#116167=DIRECTION('center_axis',(-1.4081690688991E-16,0.,-1.));
#116168=DIRECTION('ref_axis',(-1.,0.,1.13676889660403E-16));
#116169=DIRECTION('center_axis',(-0.978360123517642,0.206909324620909,-9.77058627110058E-6));
#116170=DIRECTION('ref_axis',(0.180976161286485,0.855713599897814,-0.484769908302827));
#116171=DIRECTION('center_axis',(0.994414268361317,-0.105547443284825,-9.77051739609162E-6));
#116172=DIRECTION('ref_axis',(0.0923122812911824,0.869764184940213,-0.484756336026775));
#116173=DIRECTION('center_axis',(-1.4081690688991E-16,0.,-1.));
#116174=DIRECTION('ref_axis',(-1.,0.,1.15974593313694E-16));
#116175=DIRECTION('center_axis',(0.977604079204551,-0.210452521944373,1.81624797413809E-5));
#116176=DIRECTION('ref_axis',(0.182084057578138,0.845868804767363,0.501349539839535));
#116177=DIRECTION('center_axis',(-0.994790133859856,0.101944049587673,1.81316451772609E-5));
#116178=DIRECTION('ref_axis',(0.0883925913426408,0.862463698459305,0.49834036424479));
#116179=DIRECTION('center_axis',(-1.4081690688991E-16,0.,-1.));
#116180=DIRECTION('ref_axis',(-1.,0.,1.16261524579732E-16));
#116181=DIRECTION('center_axis',(0.977601235481153,-0.210465731281114,1.84940604206757E-5));
#116182=DIRECTION('ref_axis',(0.182479018596279,0.847560772124483,-0.498339387694661));
#116183=DIRECTION('center_axis',(-0.99479151117877,0.101930608471928,1.85257116294611E-5));
#116184=DIRECTION('ref_axis',(0.0881857549144201,0.860739767464283,-0.50134850686494));
#116185=DIRECTION('center_axis',(-1.4081690688991E-16,0.,-1.));
#116186=DIRECTION('ref_axis',(-1.,0.,1.40816906889911E-16));
#116187=DIRECTION('center_axis',(-1.4081690688991E-16,0.,-1.));
#116188=DIRECTION('ref_axis',(-1.,0.,1.4081690688991E-16));
#116189=DIRECTION('',(-0.104528463267657,-0.994521895368273,1.47193748793071E-17));
#116190=DIRECTION('center_axis',(-1.4081690688991E-16,0.,-1.));
#116191=DIRECTION('ref_axis',(-1.,0.,1.4081690688991E-16));
#116192=DIRECTION('center_axis',(-1.4081690688991E-16,0.,-1.));
#116193=DIRECTION('ref_axis',(-1.,0.,1.4081690688991E-16));
#116194=DIRECTION('center_axis',(-1.4081690688991E-16,0.,-1.));
#116195=DIRECTION('ref_axis',(-1.,0.,1.4081690688991E-16));
#116196=DIRECTION('',(3.49148133884313E-15,1.,-4.91659602599733E-31));
#116197=DIRECTION('center_axis',(1.4081690688991E-16,0.,1.));
#116198=DIRECTION('ref_axis',(1.,0.,-1.4081690688991E-16));
#116199=DIRECTION('',(-0.0522695260941986,-0.497265611060785,0.866022406579779));
#116200=DIRECTION('center_axis',(1.4081690688991E-16,0.,1.));
#116201=DIRECTION('ref_axis',(-1.,0.,1.40816906889911E-16));
#116202=DIRECTION('',(-4.77800116381153E-6,0.500005191252011,-0.866022406579767));
#116203=DIRECTION('center_axis',(-1.4081690688991E-16,0.,-1.));
#116204=DIRECTION('ref_axis',(-1.,0.,1.40816906889911E-16));
#116205=DIRECTION('center_axis',(-1.4081690688991E-16,0.,-1.));
#116206=DIRECTION('ref_axis',(-1.,0.,1.4081690688991E-16));
#116207=DIRECTION('',(-0.104528463267657,-0.994521895368273,1.47193748793071E-17));
#116208=DIRECTION('center_axis',(1.4081690688991E-16,0.,1.));
#116209=DIRECTION('ref_axis',(-1.,0.,1.4081690688991E-16));
#116210=DIRECTION('',(3.49148133884313E-15,1.,-4.91659602599733E-31));
#116211=DIRECTION('center_axis',(-1.4081690688991E-16,0.,-1.));
#116212=DIRECTION('ref_axis',(-1.,0.,1.4081690688991E-16));
#116213=DIRECTION('center_axis',(-1.4081690688991E-16,0.,-1.));
#116214=DIRECTION('ref_axis',(1.,0.,-1.4081690688991E-16));
#116215=DIRECTION('',(-0.0522601510654385,-0.497266395846527,-0.866022521746648));
#116216=DIRECTION('center_axis',(-1.4081690688991E-16,0.,-1.));
#116217=DIRECTION('ref_axis',(-1.,0.,1.4081690688991E-16));
#116218=DIRECTION('center_axis',(-1.4081690688991E-16,0.,-1.));
#116219=DIRECTION('ref_axis',(-1.,0.,1.4081690688991E-16));
#116220=DIRECTION('center_axis',(-1.4081690688991E-16,0.,-1.));
#116221=DIRECTION('ref_axis',(-1.,0.,1.4081690688991E-16));
#116222=DIRECTION('',(4.62770265447403E-6,0.500004991781227,0.866022521746657));
#116223=DIRECTION('center_axis',(-1.4081690688991E-16,0.,-1.));
#116224=DIRECTION('ref_axis',(-1.,0.,1.40816906889911E-16));
#116225=DIRECTION('',(-0.104528463267657,-0.994521895368273,1.47193748793071E-17));
#116226=DIRECTION('center_axis',(1.4081690688991E-16,0.,1.));
#116227=DIRECTION('ref_axis',(-1.,0.,1.4081690688991E-16));
#116228=DIRECTION('',(3.49148133884313E-15,1.,-4.91659602599733E-31));
#116229=DIRECTION('center_axis',(-1.4081690688991E-16,0.,-1.));
#116230=DIRECTION('ref_axis',(-1.,0.,1.17174841180864E-16));
#116231=DIRECTION('center_axis',(-0.994633197962182,0.103464010407828,7.86457203065501E-6));
#116232=DIRECTION('ref_axis',(-7.97390954032785E-6,-6.43152300427559E-7,
-0.999999999968002));
#116233=DIRECTION('center_axis',(0.999999427244995,-0.00107025596491175,
7.86457225179323E-6));
#116234=DIRECTION('ref_axis',(0.000911792658825042,0.848044334090874,-0.529924500330484));
#116235=DIRECTION('center_axis',(-1.4081690688991E-16,0.,-1.));
#116236=DIRECTION('ref_axis',(-1.,0.,1.13676889660403E-16));
#116237=DIRECTION('center_axis',(-0.994628478131894,0.103509373457517,-9.77058669981437E-6));
#116238=DIRECTION('ref_axis',(0.090538327344489,0.869943071289052,-0.48476990830479));
#116239=DIRECTION('center_axis',(0.999999475000345,-0.00102464802303281,
-9.77051625719004E-6));
#116240=DIRECTION('ref_axis',(0.000891471298433248,0.87464878663446,-0.484756336026452));
#116241=DIRECTION('center_axis',(-1.4081690688991E-16,0.,-1.));
#116242=DIRECTION('ref_axis',(-1.,0.,1.15974593313694E-16));
#116243=DIRECTION('center_axis',(0.994246940479906,-0.107112188925774,1.81624797806968E-5));
#116244=DIRECTION('ref_axis',(0.0926692157705482,0.860268013673723,0.501349539840557));
#116245=DIRECTION('center_axis',(-0.999996624262643,-0.00259829454878502,
1.81316452283592E-5));
#116246=DIRECTION('ref_axis',(0.00224363754549732,-0.86697857381378,-0.498340364247558));
#116247=DIRECTION('center_axis',(-1.4081690688991E-16,0.,-1.));
#116248=DIRECTION('ref_axis',(-1.,0.,1.16261524579732E-16));
#116249=DIRECTION('center_axis',(0.994245493086383,-0.107125623150506,1.84940601461275E-5));
#116250=DIRECTION('ref_axis',(0.0928851544031254,0.861991996924917,-0.498339387695677));
#116251=DIRECTION('center_axis',(-0.999996589057285,-0.00261180600212912,
1.85257108423049E-5));
#116252=DIRECTION('ref_axis',(0.0022691410444307,-0.865242466404122,0.501348506859083));
#116253=DIRECTION('center_axis',(-1.4081690688991E-16,0.,-1.));
#116254=DIRECTION('ref_axis',(-1.,0.,1.40816906889911E-16));
#116255=DIRECTION('center_axis',(-1.4081690688991E-16,0.,-1.));
#116256=DIRECTION('ref_axis',(-1.,0.,1.4081690688991E-16));
#116257=DIRECTION('',(-3.49148133884313E-15,-1.,4.91659602599733E-31));
#116258=DIRECTION('center_axis',(-1.4081690688991E-16,0.,-1.));
#116259=DIRECTION('ref_axis',(-1.,0.,1.4081690688991E-16));
#116260=DIRECTION('center_axis',(-1.4081690688991E-16,0.,-1.));
#116261=DIRECTION('ref_axis',(-1.,0.,1.4081690688991E-16));
#116262=DIRECTION('center_axis',(-1.4081690688991E-16,0.,-1.));
#116263=DIRECTION('ref_axis',(-1.,0.,1.4081690688991E-16));
#116264=DIRECTION('',(-0.10452846326765,0.994521895368274,1.47193748793061E-17));
#116265=DIRECTION('center_axis',(1.4081690688991E-16,0.,1.));
#116266=DIRECTION('ref_axis',(1.,0.,-1.4081690688991E-16));
#116267=DIRECTION('',(-4.77800116722343E-6,-0.500005191252011,0.866022406579767));
#116268=DIRECTION('center_axis',(1.4081690688991E-16,0.,1.));
#116269=DIRECTION('ref_axis',(-1.,0.,1.40816906889911E-16));
#116270=DIRECTION('',(-0.0522695260941986,0.497265611060785,-0.866022406579779));
#116271=DIRECTION('center_axis',(-1.4081690688991E-16,0.,-1.));
#116272=DIRECTION('ref_axis',(-1.,0.,1.40816906889911E-16));
#116273=DIRECTION('center_axis',(-1.4081690688991E-16,0.,-1.));
#116274=DIRECTION('ref_axis',(-1.,0.,1.4081690688991E-16));
#116275=DIRECTION('',(-3.49148133884313E-15,-1.,4.91659602599733E-31));
#116276=DIRECTION('center_axis',(1.4081690688991E-16,0.,1.));
#116277=DIRECTION('ref_axis',(-1.,0.,1.4081690688991E-16));
#116278=DIRECTION('',(-0.10452846326765,0.994521895368274,1.47193748793061E-17));
#116279=DIRECTION('center_axis',(-1.4081690688991E-16,0.,-1.));
#116280=DIRECTION('ref_axis',(-1.,0.,1.4081690688991E-16));
#116281=DIRECTION('center_axis',(-1.4081690688991E-16,0.,-1.));
#116282=DIRECTION('ref_axis',(1.,0.,-1.4081690688991E-16));
#116283=DIRECTION('',(4.62770265084889E-6,-0.500004991781227,-0.866022521746657));
#116284=DIRECTION('center_axis',(-1.4081690688991E-16,0.,-1.));
#116285=DIRECTION('ref_axis',(-1.,0.,1.4081690688991E-16));
#116286=DIRECTION('center_axis',(-1.4081690688991E-16,0.,-1.));
#116287=DIRECTION('ref_axis',(-1.,0.,1.4081690688991E-16));
#116288=DIRECTION('center_axis',(-1.4081690688991E-16,0.,-1.));
#116289=DIRECTION('ref_axis',(-1.,0.,1.4081690688991E-16));
#116290=DIRECTION('',(-0.0522601510654331,0.497266395846486,0.866022521746671));
#116291=DIRECTION('center_axis',(-1.4081690688991E-16,0.,-1.));
#116292=DIRECTION('ref_axis',(-1.,0.,1.40816906889911E-16));
#116293=DIRECTION('',(-3.49148133884313E-15,-1.,4.91659602599733E-31));
#116294=DIRECTION('center_axis',(1.4081690688991E-16,0.,1.));
#116295=DIRECTION('ref_axis',(-1.,0.,1.4081690688991E-16));
#116296=DIRECTION('',(-0.10452846326765,0.994521895368274,1.47193748793061E-17));
#116297=DIRECTION('center_axis',(-1.4081690688991E-16,0.,-1.));
#116298=DIRECTION('ref_axis',(-1.,0.,1.17174841180864E-16));
#116299=DIRECTION('center_axis',(-0.999999427244995,-0.0010702559647792,
7.86457202574355E-6));
#116300=DIRECTION('ref_axis',(-7.86299990339083E-6,-1.47312957758963E-6,
-0.999999999968002));
#116301=DIRECTION('center_axis',(0.994633197962196,0.103464010407699,7.86457225586277E-6));
#116302=DIRECTION('ref_axis',(-0.0877379732621213,0.843493966781849,-0.52992450033045));
#116303=DIRECTION('center_axis',(-1.4081690688991E-16,0.,-1.));
#116304=DIRECTION('ref_axis',(-1.,0.,1.13676889660403E-16));
#116305=DIRECTION('center_axis',(-0.999999475000305,-0.00102464806168893,
-9.77058600784865E-6));
#116306=DIRECTION('ref_axis',(0.00089146345812007,-0.874641264345843,0.484769908303318));
#116307=DIRECTION('center_axis',(0.994628478127861,0.103509373496281,-9.77051628788904E-6));
#116308=DIRECTION('ref_axis',(0.0905391058403898,-0.869950553189685,0.484756336027271));
#116309=DIRECTION('center_axis',(-1.4081690688991E-16,0.,-1.));
#116310=DIRECTION('ref_axis',(-1.,0.,1.15974593313694E-16));
#116311=DIRECTION('center_axis',(0.999996624215829,-0.00259831235053714,
1.81624797955926E-5));
#116312=DIRECTION('ref_axis',(0.00223907064273736,0.865241946196868,0.501349539846316));
#116313=DIRECTION('center_axis',(-0.994246942387256,-0.107112171226408,
1.81316452589115E-5));
#116314=DIRECTION('ref_axis',(0.0928552846706877,-0.861994650485332,-0.498340364252582));
#116315=DIRECTION('center_axis',(-1.4081690688991E-16,0.,-1.));
#116316=DIRECTION('ref_axis',(-1.,0.,1.16261524579732E-16));
#116317=DIRECTION('center_axis',(0.999996589010145,-0.00261182427511404,
1.84940600372377E-5));
#116318=DIRECTION('ref_axis',(0.00227362102100041,0.866979057022621,-0.498339387698403));
#116319=DIRECTION('center_axis',(-0.994245495043456,-0.107125604981216,
1.85257132984629E-5));
#116320=DIRECTION('ref_axis',(0.0926991758193393,-0.86026538781347,0.501348506861799));
#116321=DIRECTION('center_axis',(-1.4081690688991E-16,0.,-1.));
#116322=DIRECTION('ref_axis',(-1.,0.,1.40816906889911E-16));
#116323=DIRECTION('center_axis',(-1.4081690688991E-16,0.,-1.));
#116324=DIRECTION('ref_axis',(-1.,0.,1.4081690688991E-16));
#116325=DIRECTION('',(0.10452846326765,-0.994521895368274,-1.47193748793061E-17));
#116326=DIRECTION('center_axis',(-1.4081690688991E-16,0.,-1.));
#116327=DIRECTION('ref_axis',(-1.,0.,1.4081690688991E-16));
#116328=DIRECTION('center_axis',(-1.4081690688991E-16,0.,-1.));
#116329=DIRECTION('ref_axis',(-1.,0.,1.4081690688991E-16));
#116330=DIRECTION('center_axis',(-1.4081690688991E-16,0.,-1.));
#116331=DIRECTION('ref_axis',(-1.,0.,1.4081690688991E-16));
#116332=DIRECTION('',(-0.207911690817756,0.978147600733806,2.92774812072079E-17));
#116333=DIRECTION('center_axis',(1.4081690688991E-16,0.,1.));
#116334=DIRECTION('ref_axis',(1.,0.,-1.4081690688991E-16));
#116335=DIRECTION('',(0.0522600224406464,-0.497266609935041,0.866022406579769));
#116336=DIRECTION('center_axis',(1.4081690688991E-16,0.,1.));
#116337=DIRECTION('ref_axis',(-1.,0.,1.40816906889911E-16));
#116338=DIRECTION('',(-0.103961598321248,0.489077884775271,-0.866022406579783));
#116339=DIRECTION('center_axis',(-1.4081690688991E-16,0.,-1.));
#116340=DIRECTION('ref_axis',(-1.,0.,1.40816906889911E-16));
#116341=DIRECTION('center_axis',(-1.4081690688991E-16,0.,-1.));
#116342=DIRECTION('ref_axis',(-1.,0.,1.4081690688991E-16));
#116343=DIRECTION('',(0.10452846326765,-0.994521895368274,-1.47193748793061E-17));
#116344=DIRECTION('center_axis',(1.4081690688991E-16,0.,1.));
#116345=DIRECTION('ref_axis',(-1.,0.,1.4081690688991E-16));
#116346=DIRECTION('',(-0.207911690817756,0.978147600733806,2.92774812072079E-17));
#116347=DIRECTION('center_axis',(-1.4081690688991E-16,0.,-1.));
#116348=DIRECTION('ref_axis',(-1.,0.,1.4081690688991E-16));
#116349=DIRECTION('center_axis',(-1.4081690688991E-16,0.,-1.));
#116350=DIRECTION('ref_axis',(1.,0.,-1.4081690688991E-16));
#116351=DIRECTION('',(0.0522693557686642,-0.497265428393217,-0.866022521746657));
#116352=DIRECTION('center_axis',(-1.4081690688991E-16,0.,-1.));
#116353=DIRECTION('ref_axis',(-1.,0.,1.4081690688991E-16));
#116354=DIRECTION('center_axis',(-1.4081690688991E-16,0.,-1.));
#116355=DIRECTION('ref_axis',(-1.,0.,1.4081690688991E-16));
#116356=DIRECTION('center_axis',(-1.4081690688991E-16,0.,-1.));
#116357=DIRECTION('ref_axis',(-1.,0.,1.4081690688991E-16));
#116358=DIRECTION('',(-0.103952356682315,0.489079645219204,0.866022521746664));
#116359=DIRECTION('center_axis',(-1.4081690688991E-16,0.,-1.));
#116360=DIRECTION('ref_axis',(-1.,0.,1.40816906889911E-16));
#116361=DIRECTION('',(0.10452846326765,-0.994521895368274,-1.47193748793061E-17));
#116362=DIRECTION('center_axis',(1.4081690688991E-16,0.,1.));
#116363=DIRECTION('ref_axis',(-1.,0.,1.4081690688991E-16));
#116364=DIRECTION('',(-0.207911690817756,0.978147600733806,2.92774812072079E-17));
#116365=DIRECTION('center_axis',(-1.4081690688991E-16,0.,-1.));
#116366=DIRECTION('ref_axis',(-1.,0.,1.17174841180864E-16));
#116367=DIRECTION('center_axis',(-0.99440945353958,-0.105592796389066,7.86457201556077E-6));
#116368=DIRECTION('ref_axis',(-7.66594159182268E-6,-2.28696686047188E-6,
-0.999999999968001));
#116369=DIRECTION('center_axis',(0.978369559222142,0.20686470343106,7.86457223501791E-6));
#116370=DIRECTION('ref_axis',(-0.175426463587678,0.829702103060261,-0.529924500330472));
#116371=DIRECTION('center_axis',(-1.4081690688991E-16,0.,-1.));
#116372=DIRECTION('ref_axis',(-1.,0.,1.13676889660403E-16));
#116373=DIRECTION('center_axis',(-0.994414268357372,-0.105547443321989,
-9.77058482928466E-6));
#116374=DIRECTION('ref_axis',(0.0923114872004343,-0.869756704677923,0.484769908305625));
#116375=DIRECTION('center_axis',(0.978360123509597,0.206909324658953,-9.7705160822993E-6));
#116376=DIRECTION('ref_axis',(0.180977717589175,-0.855720959436191,0.484756336026481));
#116377=DIRECTION('center_axis',(-1.4081690688991E-16,0.,-1.));
#116378=DIRECTION('ref_axis',(-1.,0.,1.15974593313694E-16));
#116379=DIRECTION('center_axis',(0.99479013567409,0.101944031878529,1.81624797615794E-5));
#116380=DIRECTION('ref_axis',(0.0882156062113998,-0.860736106899266,-0.501349539842862));
#116381=DIRECTION('center_axis',(-0.977604082951519,-0.210452504541434,
1.81316453016117E-5));
#116382=DIRECTION('ref_axis',(0.182449589865665,-0.847566533384306,-0.498340364253952));
#116383=DIRECTION('center_axis',(-1.4081690688991E-16,0.,-1.));
#116384=DIRECTION('ref_axis',(-1.,0.,1.16261524579732E-16));
#116385=DIRECTION('center_axis',(0.994791513041743,0.101930590295988,1.8494064067236E-5));
#116386=DIRECTION('ref_axis',(0.0883628226286463,-0.862467313145872,0.498339387698825));
#116387=DIRECTION('center_axis',(-0.977601239327261,-0.210465713413377,
1.85257180944615E-5));
#116388=DIRECTION('ref_axis',(0.182113579025377,-0.845863061613112,0.501348506862303));
#116389=DIRECTION('center_axis',(-1.4081690688991E-16,0.,-1.));
#116390=DIRECTION('ref_axis',(-1.,0.,1.40816906889911E-16));
#116391=DIRECTION('center_axis',(-1.4081690688991E-16,0.,-1.));
#116392=DIRECTION('ref_axis',(-1.,0.,1.4081690688991E-16));
#116393=DIRECTION('',(0.207911690817756,-0.978147600733806,-2.92774812072079E-17));
#116394=DIRECTION('center_axis',(-1.4081690688991E-16,0.,-1.));
#116395=DIRECTION('ref_axis',(-1.,0.,1.4081690688991E-16));
#116396=DIRECTION('center_axis',(-1.4081690688991E-16,0.,-1.));
#116397=DIRECTION('ref_axis',(-1.,0.,1.4081690688991E-16));
#116398=DIRECTION('center_axis',(-1.4081690688991E-16,0.,-1.));
#116399=DIRECTION('ref_axis',(-1.,0.,1.4081690688991E-16));
#116400=DIRECTION('',(-0.309016994374945,0.951056516295154,4.35148173242966E-17));
#116401=DIRECTION('center_axis',(1.4081690688991E-16,0.,1.));
#116402=DIRECTION('ref_axis',(1.,0.,-1.4081690688991E-16));
#116403=DIRECTION('',(0.103952251140481,-0.489079871579878,0.866022406579781));
#116404=DIRECTION('center_axis',(1.4081690688991E-16,0.,1.));
#116405=DIRECTION('ref_axis',(-1.,0.,1.40816906889911E-16));
#116406=DIRECTION('',(-0.154514645521691,0.475531718838031,-0.866022406579792));
#116407=DIRECTION('center_axis',(-1.4081690688991E-16,0.,-1.));
#116408=DIRECTION('ref_axis',(-1.,0.,1.40816906889911E-16));
#116409=DIRECTION('center_axis',(-1.4081690688991E-16,0.,-1.));
#116410=DIRECTION('ref_axis',(-1.,0.,1.4081690688991E-16));
#116411=DIRECTION('',(0.207911690817756,-0.978147600733806,-2.92774812072079E-17));
#116412=DIRECTION('center_axis',(1.4081690688991E-16,0.,1.));
#116413=DIRECTION('ref_axis',(-1.,0.,1.4081690688991E-16));
#116414=DIRECTION('',(-0.309016994374945,0.951056516295154,4.35148173242966E-17));
#116415=DIRECTION('center_axis',(-1.4081690688991E-16,0.,-1.));
#116416=DIRECTION('ref_axis',(-1.,0.,1.4081690688991E-16));
#116417=DIRECTION('center_axis',(-1.4081690688991E-16,0.,-1.));
#116418=DIRECTION('ref_axis',(1.,0.,-1.4081690688991E-16));
#116419=DIRECTION('',(0.103961409834804,-0.489077720912242,-0.866022521746662));
#116420=DIRECTION('center_axis',(-1.4081690688991E-16,0.,-1.));
#116421=DIRECTION('ref_axis',(-1.,0.,1.4081690688991E-16));
#116422=DIRECTION('center_axis',(-1.4081690688991E-16,0.,-1.));
#116423=DIRECTION('ref_axis',(-1.,0.,1.4081690688991E-16));
#116424=DIRECTION('center_axis',(-1.4081690688991E-16,0.,-1.));
#116425=DIRECTION('ref_axis',(-1.,0.,1.4081690688991E-16));
#116426=DIRECTION('',(-0.154505638525963,0.475534435652421,0.866022521746645));
#116427=DIRECTION('center_axis',(-1.4081690688991E-16,0.,-1.));
#116428=DIRECTION('ref_axis',(-1.,0.,1.40816906889911E-16));
#116429=DIRECTION('',(0.207911690817756,-0.978147600733806,-2.92774812072079E-17));
#116430=DIRECTION('center_axis',(1.4081690688991E-16,0.,1.));
#116431=DIRECTION('ref_axis',(-1.,0.,1.4081690688991E-16));
#116432=DIRECTION('',(-0.309016994374945,0.951056516295154,4.35148173242966E-17));
#116433=DIRECTION('center_axis',(-1.4081690688991E-16,0.,-1.));
#116434=DIRECTION('ref_axis',(-1.,0.,1.17174841180864E-16));
#116435=DIRECTION('center_axis',(-0.977924521767625,-0.208958440039425,
7.86457203496813E-6));
#116436=DIRECTION('ref_axis',(-7.38489364321875E-6,-3.07574773432254E-6,
-0.999999999968002));
#116437=DIRECTION('center_axis',(0.95138669885428,0.307998943474332,7.86457235843123E-6));
#116438=DIRECTION('ref_axis',(-0.261192944867685,0.806819849471268,-0.529924500330478));
#116439=DIRECTION('center_axis',(-1.4081690688991E-16,0.,-1.));
#116440=DIRECTION('ref_axis',(-1.,0.,1.13676889660403E-16));
#116441=DIRECTION('center_axis',(-0.977934050895729,-0.208913838706787,
-9.77058511661614E-6));
#116442=DIRECTION('ref_axis',(0.182720126971744,-0.855342908547616,0.484769908303655));
#116443=DIRECTION('center_axis',(0.951372650643379,0.308042333961304,-9.77051741258055E-6));
#116444=DIRECTION('ref_axis',(0.269433499591897,-0.832115907779229,0.484756336027093));
#116445=DIRECTION('center_axis',(-1.4081690688991E-16,0.,-1.));
#116446=DIRECTION('ref_axis',(-1.,0.,1.15974593313694E-16));
#116447=DIRECTION('center_axis',(0.9786845182327,0.205369455961084,1.8162479768661E-5));
#116448=DIRECTION('ref_axis',(0.177703774422995,-0.846799862689322,-0.501349539847368));
#116449=DIRECTION('center_axis',(-0.95025038860616,-0.311487076176663,1.81316453262635E-5));
#116450=DIRECTION('ref_axis',(0.270044939174518,-0.823852299980834,-0.498340364251704));
#116451=DIRECTION('center_axis',(-1.4081690688991E-16,0.,-1.));
#116452=DIRECTION('ref_axis',(-1.,0.,1.16261524579732E-16));
#116453=DIRECTION('center_axis',(0.978687293082516,0.205356231989163,1.84940676879274E-5));
#116454=DIRECTION('ref_axis',(0.178031144703038,-0.848506196906464,0.498339387693823));
#116455=DIRECTION('center_axis',(-0.950246179854085,-0.311499915456677,
1.85257046986954E-5));
#116456=DIRECTION('ref_axis',(0.269532707750914,-0.822193282704966,0.501348506856551));
#116457=DIRECTION('center_axis',(-1.4081690688991E-16,0.,-1.));
#116458=DIRECTION('ref_axis',(-1.,0.,1.40816906889911E-16));
#116459=DIRECTION('center_axis',(-1.4081690688991E-16,0.,-1.));
#116460=DIRECTION('ref_axis',(-1.,0.,1.4081690688991E-16));
#116461=DIRECTION('',(0.309016994374945,-0.951056516295154,-4.35148173242966E-17));
#116462=DIRECTION('center_axis',(-1.4081690688991E-16,0.,-1.));
#116463=DIRECTION('ref_axis',(-1.,0.,1.4081690688991E-16));
#116464=DIRECTION('center_axis',(-1.4081690688991E-16,0.,-1.));
#116465=DIRECTION('ref_axis',(-1.,0.,1.4081690688991E-16));
#116466=DIRECTION('center_axis',(-1.4081690688991E-16,0.,-1.));
#116467=DIRECTION('ref_axis',(-1.,0.,1.4081690688991E-16));
#116468=DIRECTION('',(-0.406736643075798,0.913545457642602,5.72753959967194E-17));
#116469=DIRECTION('center_axis',(1.4081690688991E-16,0.,1.));
#116470=DIRECTION('ref_axis',(1.,0.,-1.4081690688991E-16));
#116471=DIRECTION('',(0.154505557223429,-0.475534671805166,0.866022406579778));
#116472=DIRECTION('center_axis',(1.4081690688991E-16,0.,1.));
#116473=DIRECTION('ref_axis',(-1.,0.,1.40816906889911E-16));
#116474=DIRECTION('',(-0.20337479793158,0.456775527877825,-0.866022406579774));
#116475=DIRECTION('center_axis',(-1.4081690688991E-16,0.,-1.));
#116476=DIRECTION('ref_axis',(-1.,0.,1.40816906889911E-16));
#116477=DIRECTION('center_axis',(-1.4081690688991E-16,0.,-1.));
#116478=DIRECTION('ref_axis',(-1.,0.,1.4081690688991E-16));
#116479=DIRECTION('',(0.309016994374945,-0.951056516295154,-4.35148173242966E-17));
#116480=DIRECTION('center_axis',(1.4081690688991E-16,0.,1.));
#116481=DIRECTION('ref_axis',(-1.,0.,1.4081690688991E-16));
#116482=DIRECTION('',(-0.406736643075798,0.913545457642602,5.72753959967194E-17));
#116483=DIRECTION('center_axis',(-1.4081690688991E-16,0.,-1.));
#116484=DIRECTION('ref_axis',(-1.,0.,1.4081690688991E-16));
#116485=DIRECTION('center_axis',(-1.4081690688991E-16,0.,-1.));
#116486=DIRECTION('ref_axis',(1.,0.,-1.4081690688991E-16));
#116487=DIRECTION('',(0.154514440939481,-0.475531575574859,-0.866022521746664));
#116488=DIRECTION('center_axis',(-1.4081690688991E-16,0.,-1.));
#116489=DIRECTION('ref_axis',(-1.,0.,1.4081690688991E-16));
#116490=DIRECTION('center_axis',(-1.4081690688991E-16,0.,-1.));
#116491=DIRECTION('ref_axis',(-1.,0.,1.4081690688991E-16));
#116492=DIRECTION('center_axis',(-1.4081690688991E-16,0.,-1.));
#116493=DIRECTION('ref_axis',(-1.,0.,1.4081690688991E-16));
#116494=DIRECTION('',(-0.203366124261491,0.456779171296611,0.866022521746658));
#116495=DIRECTION('center_axis',(-1.4081690688991E-16,0.,-1.));
#116496=DIRECTION('ref_axis',(-1.,0.,1.40816906889911E-16));
#116497=DIRECTION('',(0.309016994374945,-0.951056516295154,-4.35148173242966E-17));
#116498=DIRECTION('center_axis',(1.4081690688991E-16,0.,1.));
#116499=DIRECTION('ref_axis',(-1.,0.,1.4081690688991E-16));
#116500=DIRECTION('',(-0.406736643075798,0.913545457642602,5.72753959967194E-17));
#116501=DIRECTION('center_axis',(-1.4081690688991E-16,0.,-1.));
#116502=DIRECTION('ref_axis',(-1.,0.,1.17174841180864E-16));
#116503=DIRECTION('center_axis',(-0.950725244291327,-0.310034691293322,
7.86457203087576E-6));
#116504=DIRECTION('ref_axis',(-7.02293522902363E-6,-3.83083008160136E-6,
-0.999999999968002));
#116505=DIRECTION('center_axis',(0.913980246723271,0.405758682640085,7.86457225348564E-6));
#116506=DIRECTION('ref_axis',(-0.344097741585782,0.775097908773498,-0.529924500330485));
#116507=DIRECTION('center_axis',(-1.4081690688991E-16,0.,-1.));
#116508=DIRECTION('ref_axis',(-1.,0.,1.13676889660403E-16));
#116509=DIRECTION('center_axis',(-0.950739383327519,-0.309991330353843,
-9.77057985364929E-6));
#116510=DIRECTION('ref_axis',(0.271126846795285,-0.83155779651819,0.484769908303578));
#116511=DIRECTION('center_axis',(0.913961739929036,0.405800366991488,-9.77051738652309E-6));
#116512=DIRECTION('ref_axis',(0.354937311790829,-0.799394020106138,0.484756336025892));
#116513=DIRECTION('center_axis',(-1.4081690688991E-16,0.,-1.));
#116514=DIRECTION('ref_axis',(-1.,0.,1.15974593313694E-16));
#116515=DIRECTION('center_axis',(0.951856228406623,0.306544809307943,1.81624797519335E-5));
#116516=DIRECTION('ref_axis',(0.265244982896516,-0.823585901985291,-0.501349539841518));
#116517=DIRECTION('center_axis',(-0.912485552150575,-0.409108930222384,
1.81316452567651E-5));
#116518=DIRECTION('ref_axis',(0.354681619619182,-0.791111768375823,-0.498340364250771));
#116519=DIRECTION('center_axis',(-1.4081690688991E-16,0.,-1.));
#116520=DIRECTION('ref_axis',(-1.,0.,1.16261524579732E-16));
#116521=DIRECTION('center_axis',(0.951860370338612,0.306531947824057,1.84940585634574E-5));
#116522=DIRECTION('ref_axis',(0.265748920299228,-0.825248669206012,0.498339387700291));
#116523=DIRECTION('center_axis',(-0.912480024382915,-0.409121259236127,
1.85256990113859E-5));
#116524=DIRECTION('ref_axis',(0.353998779725528,-0.789515382131506,0.501348506859828));
#116525=DIRECTION('center_axis',(-1.4081690688991E-16,0.,-1.));
#116526=DIRECTION('ref_axis',(-1.,0.,1.40816906889911E-16));
#116527=DIRECTION('center_axis',(-1.4081690688991E-16,0.,-1.));
#116528=DIRECTION('ref_axis',(-1.,0.,1.4081690688991E-16));
#116529=DIRECTION('',(0.406736643075798,-0.913545457642602,-5.72753959967194E-17));
#116530=DIRECTION('center_axis',(-1.4081690688991E-16,0.,-1.));
#116531=DIRECTION('ref_axis',(-1.,0.,1.4081690688991E-16));
#116532=DIRECTION('center_axis',(-1.4081690688991E-16,0.,-1.));
#116533=DIRECTION('ref_axis',(-1.,0.,1.4081690688991E-16));
#116534=DIRECTION('center_axis',(-1.4081690688991E-16,0.,-1.));
#116535=DIRECTION('ref_axis',(-1.,0.,1.4081690688991E-16));
#116536=DIRECTION('',(-0.499999999999998,0.86602540378444,7.04084534449549E-17));
#116537=DIRECTION('center_axis',(1.4081690688991E-16,0.,1.));
#116538=DIRECTION('ref_axis',(1.,0.,-1.4081690688991E-16));
#116539=DIRECTION('',(0.203366068089046,-0.45677941465413,0.866022406579779));
#116540=DIRECTION('center_axis',(1.4081690688991E-16,0.,1.));
#116541=DIRECTION('ref_axis',(-1.,5.32907051820075E-15,1.40816906889911E-16));
#116542=DIRECTION('',(-0.250006733496382,0.433014808647711,-0.866022406579792));
#116543=DIRECTION('center_axis',(-1.4081690688991E-16,0.,-1.));
#116544=DIRECTION('ref_axis',(-1.,0.,1.40816906889911E-16));
#116545=DIRECTION('center_axis',(-1.4081690688991E-16,0.,-1.));
#116546=DIRECTION('ref_axis',(-1.,0.,1.4081690688991E-16));
#116547=DIRECTION('',(0.406736643075798,-0.913545457642602,-5.72753959967194E-17));
#116548=DIRECTION('center_axis',(1.4081690688991E-16,0.,1.));
#116549=DIRECTION('ref_axis',(-1.,-4.44089209850063E-15,1.4081690688991E-16));
#116550=DIRECTION('',(-0.499999999999998,0.86602540378444,7.04084534449549E-17));
#116551=DIRECTION('center_axis',(-1.4081690688991E-16,0.,-1.));
#116552=DIRECTION('ref_axis',(-1.,0.,1.4081690688991E-16));
#116553=DIRECTION('center_axis',(-1.4081690688991E-16,0.,-1.));
#116554=DIRECTION('ref_axis',(1.,0.,-1.4081690688991E-16));
#116555=DIRECTION('',(0.203374579494982,-0.456775406784115,-0.866022521746661));
#116556=DIRECTION('center_axis',(-1.4081690688991E-16,0.,-1.));
#116557=DIRECTION('ref_axis',(-1.,0.,1.4081690688991E-16));
#116558=DIRECTION('center_axis',(-1.4081690688991E-16,0.,-1.));
#116559=DIRECTION('ref_axis',(-1.,0.,1.4081690688991E-16));
#116560=DIRECTION('center_axis',(-1.4081690688991E-16,0.,-1.));
#116561=DIRECTION('ref_axis',(-1.,0.,1.4081690688991E-16));
#116562=DIRECTION('',(-0.249998488182569,0.433019338752904,0.866022521746651));
#116563=DIRECTION('center_axis',(-1.4081690688991E-16,0.,-1.));
#116564=DIRECTION('ref_axis',(-1.,0.,1.40816906889911E-16));
#116565=DIRECTION('',(0.406736643075798,-0.913545457642602,-5.72753959967194E-17));
#116566=DIRECTION('center_axis',(1.4081690688991E-16,0.,1.));
#116567=DIRECTION('ref_axis',(-1.,-4.44089209850063E-15,1.4081690688991E-16));
#116568=DIRECTION('',(-0.499999999999998,0.86602540378444,7.04084534449549E-17));
#116569=DIRECTION('center_axis',(-1.4081690688991E-16,0.,-1.));
#116570=DIRECTION('ref_axis',(-1.,0.,1.17174841180864E-16));
#116571=DIRECTION('center_axis',(-0.913109622086492,-0.407714137590558,
7.86457210773485E-6));
#116572=DIRECTION('ref_axis',(-6.58403218430508E-6,-4.54394095516285E-6,
-0.999999999968001));
#116573=DIRECTION('center_axis',(0.866560035746485,0.499072844768375,7.86457220438574E-6));
#116574=DIRECTION('ref_axis',(-0.423232531439969,0.734883833187538,-0.529924500330478));
#116575=DIRECTION('center_axis',(-1.4081690688991E-16,0.,-1.));
#116576=DIRECTION('ref_axis',(-1.,0.,1.13676889660403E-16));
#116577=DIRECTION('center_axis',(-0.913128216116625,-0.407672492125978,
-9.77059469166599E-6));
#116578=DIRECTION('ref_axis',(0.356563044148412,-0.79866196325562,0.484769908303204));
#116579=DIRECTION('center_axis',(0.866537273132503,0.499112366283007,-9.77051476609031E-6));
#116580=DIRECTION('ref_axis',(0.436552356526076,-0.757913804263947,0.484756336026339));
#116581=DIRECTION('center_axis',(-1.4081690688991E-16,0.,-1.));
#116582=DIRECTION('ref_axis',(-1.,0.,1.15974593313694E-16));
#116583=DIRECTION('center_axis',(0.914599202553438,0.40436159357528,1.8162479713582E-5));
#116584=DIRECTION('ref_axis',(0.349880111830792,-0.791348561789984,-0.501349539840416));
#116585=DIRECTION('center_axis',(-0.864723333035746,-0.502248501217071,
1.8131645220716E-5));
#116586=DIRECTION('ref_axis',(0.435432334017781,-0.749703650686127,-0.498340364248894));
#116587=DIRECTION('center_axis',(-1.4081690688991E-16,0.,-1.));
#116588=DIRECTION('ref_axis',(-1.,0.,1.16261524579732E-16));
#116589=DIRECTION('center_axis',(0.914604666184872,0.404349235501724,1.84940660467886E-5));
#116590=DIRECTION('ref_axis',(0.350555095113837,-0.79294954439497,0.498339387700328));
#116591=DIRECTION('center_axis',(-0.864716546823262,-0.502260184871199,
1.85257209310319E-5));
#116592=DIRECTION('ref_axis',(0.434586366990742,-0.748187385815862,0.50134850686106));
#116593=DIRECTION('center_axis',(-1.4081690688991E-16,0.,-1.));
#116594=DIRECTION('ref_axis',(-1.,0.,1.40816906889911E-16));
#116595=DIRECTION('center_axis',(-1.4081690688991E-16,0.,-1.));
#116596=DIRECTION('ref_axis',(-1.,0.,1.4081690688991E-16));
#116597=DIRECTION('',(0.499999999999998,-0.86602540378444,-7.04084534449549E-17));
#116598=DIRECTION('center_axis',(-1.4081690688991E-16,0.,-1.));
#116599=DIRECTION('ref_axis',(-1.,0.,1.4081690688991E-16));
#116600=DIRECTION('center_axis',(-1.4081690688991E-16,0.,-1.));
#116601=DIRECTION('ref_axis',(-1.,0.,1.4081690688991E-16));
#116602=DIRECTION('center_axis',(-1.4081690688991E-16,0.,-1.));
#116603=DIRECTION('ref_axis',(-1.,0.,1.4081690688991E-16));
#116604=DIRECTION('',(-0.587785252292471,0.809016994374949,8.27701011433315E-17));
#116605=DIRECTION('center_axis',(1.4081690688991E-16,0.,1.));
#116606=DIRECTION('ref_axis',(1.,0.,-1.4081690688991E-16));
#116607=DIRECTION('',(0.249998457755605,-0.433019586648901,0.86602240657978));
#116608=DIRECTION('center_axis',(1.4081690688991E-16,0.,1.));
#116609=DIRECTION('ref_axis',(-1.,1.06581410364015E-14,1.40816906889911E-16));
#116610=DIRECTION('',(-0.293899542971745,0.404509888559929,-0.86602240657978));
#116611=DIRECTION('center_axis',(-1.4081690688991E-16,0.,-1.));
#116612=DIRECTION('ref_axis',(-1.,0.,1.40816906889911E-16));
#116613=DIRECTION('center_axis',(-1.4081690688991E-16,0.,-1.));
#116614=DIRECTION('ref_axis',(-1.,0.,1.4081690688991E-16));
#116615=DIRECTION('',(0.499999999999998,-0.86602540378444,-7.04084534449549E-17));
#116616=DIRECTION('center_axis',(1.4081690688991E-16,0.,1.));
#116617=DIRECTION('ref_axis',(-1.,0.,1.4081690688991E-16));
#116618=DIRECTION('',(-0.587785252292471,0.809016994374949,8.27701011433315E-17));
#116619=DIRECTION('center_axis',(-1.4081690688991E-16,0.,-1.));
#116620=DIRECTION('ref_axis',(-1.,0.,1.4081690688991E-16));
#116621=DIRECTION('center_axis',(-1.4081690688991E-16,0.,-1.));
#116622=DIRECTION('ref_axis',(1.,0.,-1.4081690688991E-16));
#116623=DIRECTION('',(0.250006503598675,-0.433014711050211,-0.866022521746674));
#116624=DIRECTION('center_axis',(-1.4081690688991E-16,0.,-1.));
#116625=DIRECTION('ref_axis',(-1.,0.,1.4081690688991E-16));
#116626=DIRECTION('center_axis',(-1.4081690688991E-16,0.,-1.));
#116627=DIRECTION('ref_axis',(-1.,0.,1.4081690688991E-16));
#116628=DIRECTION('center_axis',(-1.4081690688991E-16,0.,-1.));
#116629=DIRECTION('ref_axis',(-1.,0.,1.4081690688991E-16));
#116630=DIRECTION('',(-0.293891816351551,0.404515255718677,0.866022521746657));
#116631=DIRECTION('center_axis',(-1.4081690688991E-16,0.,-1.));
#116632=DIRECTION('ref_axis',(-1.,0.,1.40816906889911E-16));
#116633=DIRECTION('',(0.499999999999998,-0.86602540378444,-7.04084534449549E-17));
#116634=DIRECTION('center_axis',(1.4081690688991E-16,0.,1.));
#116635=DIRECTION('ref_axis',(-1.,0.,1.4081690688991E-16));
#116636=DIRECTION('',(-0.587785252292471,0.809016994374949,8.27701011433315E-17));
#116637=DIRECTION('center_axis',(-1.4081690688991E-16,0.,-1.));
#116638=DIRECTION('ref_axis',(-1.,0.,1.17174841180864E-16));
#116639=DIRECTION('center_axis',(-0.865489779781641,-0.50092658247659,7.86457214489057E-6));
#116640=DIRECTION('ref_axis',(-6.07299300101722E-6,-5.20726760504282E-6,
-0.999999999968002));
#116641=DIRECTION('center_axis',(0.809645611678816,0.586919060371517,7.86457245342431E-6));
#116642=DIRECTION('ref_axis',(-0.497730297112331,0.686618216541011,-0.529924500330483));
#116643=DIRECTION('center_axis',(-1.4081690688991E-16,0.,-1.));
#116644=DIRECTION('ref_axis',(-1.,0.,1.13676889660403E-16));
#116645=DIRECTION('center_axis',(-0.86551262508884,-0.500887108754418,-9.77059212653647E-6));
#116646=DIRECTION('ref_axis',(0.43809266217451,-0.75701582239318,0.484769908302101));
#116647=DIRECTION('center_axis',(0.809618842638511,0.586955986040874,-9.77051773404624E-6));
#116648=DIRECTION('ref_axis',(0.513384442288508,-0.708129726178339,0.484756336027398));
#116649=DIRECTION('center_axis',(-1.4081690688991E-16,0.,-1.));
#116650=DIRECTION('ref_axis',(-1.,0.,1.15974593313694E-16));
#116651=DIRECTION('center_axis',(0.867321636444858,0.497748107605381,1.81624797810239E-5));
#116652=DIRECTION('ref_axis',(0.430681881042823,-0.750441041151016,-0.501349539839815));
#116653=DIRECTION('center_axis',(-0.80748702412921,-0.589885332530142,1.81316451347442E-5));
#116654=DIRECTION('ref_axis',(0.511412360641924,-0.700081622909619,-0.498340364256086));
#116655=DIRECTION('center_axis',(-1.4081690688991E-16,0.,-1.));
#116656=DIRECTION('ref_axis',(-1.,0.,1.16261524579732E-16));
#116657=DIRECTION('center_axis',(0.867328361919153,0.49773638833082,1.84940564337033E-5));
#116658=DIRECTION('ref_axis',(0.431520514948347,-0.751962698440794,0.49833938769914));
#116659=DIRECTION('center_axis',(-0.807479053810967,-0.589896242837114,
1.85257006906714E-5));
#116660=DIRECTION('ref_axis',(0.510412535076058,-0.698662091933164,0.50134850686205));
#116661=DIRECTION('center_axis',(-1.4081690688991E-16,0.,-1.));
#116662=DIRECTION('ref_axis',(-1.,0.,1.40816906889911E-16));
#116663=DIRECTION('center_axis',(-1.4081690688991E-16,0.,-1.));
#116664=DIRECTION('ref_axis',(-1.,0.,1.4081690688991E-16));
#116665=DIRECTION('',(0.587785252292471,-0.809016994374949,-8.27701011433315E-17));
#116666=DIRECTION('center_axis',(-1.4081690688991E-16,0.,-1.));
#116667=DIRECTION('ref_axis',(-1.,0.,1.4081690688991E-16));
#116668=DIRECTION('center_axis',(-1.4081690688991E-16,0.,-1.));
#116669=DIRECTION('ref_axis',(-1.,0.,1.4081690688991E-16));
#116670=DIRECTION('center_axis',(-1.4081690688991E-16,0.,-1.));
#116671=DIRECTION('ref_axis',(-1.,0.,1.4081690688991E-16));
#116672=DIRECTION('',(-0.669130606358857,0.743144825477395,9.42249022928245E-17));
#116673=DIRECTION('center_axis',(1.4081690688991E-16,0.,1.));
#116674=DIRECTION('ref_axis',(1.,0.,-1.4081690688991E-16));
#116675=DIRECTION('',(0.293891812003446,-0.404515505437187,0.866022406579777));
#116676=DIRECTION('center_axis',(1.4081690688991E-16,0.,1.));
#116677=DIRECTION('ref_axis',(-1.,0.,1.40816906889911E-16));
#116678=DIRECTION('',(-0.334572327551833,0.371573073483921,-0.866022406579796));
#116679=DIRECTION('center_axis',(-1.4081690688991E-16,0.,-1.));
#116680=DIRECTION('ref_axis',(-1.,0.,1.40816906889911E-16));
#116681=DIRECTION('center_axis',(-1.4081690688991E-16,0.,-1.));
#116682=DIRECTION('ref_axis',(-1.,0.,1.4081690688991E-16));
#116683=DIRECTION('',(0.587785252292471,-0.809016994374949,-8.27701011433315E-17));
#116684=DIRECTION('center_axis',(1.4081690688991E-16,0.,1.));
#116685=DIRECTION('ref_axis',(-1.,0.,1.4081690688991E-16));
#116686=DIRECTION('',(-0.669130606358857,0.743144825477395,9.42249022928245E-17));
#116687=DIRECTION('center_axis',(-1.4081690688991E-16,0.,-1.));
#116688=DIRECTION('ref_axis',(-1.,0.,1.4081690688991E-16));
#116689=DIRECTION('center_axis',(-1.4081690688991E-16,0.,-1.));
#116690=DIRECTION('ref_axis',(1.,0.,-1.4081690688991E-16));
#116691=DIRECTION('',(0.293899304131716,-0.404509815527969,-0.866022521746647));
#116692=DIRECTION('center_axis',(-1.4081690688991E-16,0.,-1.));
#116693=DIRECTION('ref_axis',(-1.,0.,1.4081690688991E-16));
#116694=DIRECTION('center_axis',(-1.4081690688991E-16,0.,-1.));
#116695=DIRECTION('ref_axis',(-1.,0.,1.4081690688991E-16));
#116696=DIRECTION('center_axis',(-1.4081690688991E-16,0.,-1.));
#116697=DIRECTION('ref_axis',(-1.,0.,1.4081690688991E-16));
#116698=DIRECTION('',(-0.334565204279747,0.371579218892574,0.866022521746655));
#116699=DIRECTION('center_axis',(-1.4081690688991E-16,0.,-1.));
#116700=DIRECTION('ref_axis',(-1.,0.,1.40816906889911E-16));
#116701=DIRECTION('',(0.587785252292471,-0.809016994374949,-8.27701011433315E-17));
#116702=DIRECTION('center_axis',(1.4081690688991E-16,0.,1.));
#116703=DIRECTION('ref_axis',(-1.,0.,1.4081690688991E-16));
#116704=DIRECTION('',(-0.669130606358857,0.743144825477395,9.42249022928245E-17));
#116705=DIRECTION('center_axis',(-1.4081690688991E-16,0.,-1.));
#116706=DIRECTION('ref_axis',(-1.,0.,1.17174841180864E-16));
#116707=DIRECTION('center_axis',(-0.808387450334234,-0.588650770899236,
7.86457176845602E-6));
#116708=DIRECTION('ref_axis',(-5.49541649073876E-6,-5.81354209923377E-6,
-0.999999999968002));
#116709=DIRECTION('center_axis',(0.743860540860191,0.668334867928745,7.86457216966126E-6));
#116710=DIRECTION('ref_axis',(-0.566774825493195,0.630829867029678,-0.52992450033045));
#116711=DIRECTION('center_axis',(-1.4081690688991E-16,0.,-1.));
#116712=DIRECTION('ref_axis',(-1.,0.,1.13676889660403E-16));
#116713=DIRECTION('center_axis',(-0.808414296619818,-0.588613901403305,
-9.77059222526084E-6));
#116714=DIRECTION('ref_axis',(0.514822445316686,-0.707075657764177,0.484769908302387));
#116715=DIRECTION('center_axis',(0.743830058675508,0.668368793193793,-9.77050528701263E-6));
#116716=DIRECTION('ref_axis',(0.584591780669454,-0.650587230628161,0.484756336025942));
#116717=DIRECTION('center_axis',(-1.4081690688991E-16,0.,-1.));
#116718=DIRECTION('ref_axis',(-1.,0.,1.15974593313694E-16));
#116719=DIRECTION('center_axis',(0.810541512988656,0.585681189208076,1.81624796940111E-5));
#116720=DIRECTION('ref_axis',(0.506765009440592,-0.701311531425889,-0.501349539837977));
#116721=DIRECTION('center_axis',(-0.741403718408774,-0.671059256698607,
1.81316451549553E-5));
#116722=DIRECTION('ref_axis',(0.58178924642817,-0.642789354378085,-0.498340364247917));
#116723=DIRECTION('center_axis',(-1.4081690688991E-16,0.,-1.));
#116724=DIRECTION('ref_axis',(-1.,0.,1.16261524579732E-16));
#116725=DIRECTION('center_axis',(0.810549426621222,0.585670237131766,1.84940465536676E-5));
#116726=DIRECTION('ref_axis',(0.507758105721217,-0.702737191806194,0.498339387693513));
#116727=DIRECTION('center_axis',(-0.741394651320048,-0.671069274107243,
1.85257134388176E-5));
#116728=DIRECTION('ref_axis',(0.580646516618426,-0.641482109969101,0.501348506857733));
#116729=DIRECTION('center_axis',(-1.4081690688991E-16,0.,-1.));
#116730=DIRECTION('ref_axis',(-1.,0.,1.40816906889911E-16));
#116731=DIRECTION('center_axis',(-1.4081690688991E-16,0.,-1.));
#116732=DIRECTION('ref_axis',(-1.,0.,1.4081690688991E-16));
#116733=DIRECTION('',(0.669130606358857,-0.743144825477395,-9.42249022928245E-17));
#116734=DIRECTION('center_axis',(-1.4081690688991E-16,0.,-1.));
#116735=DIRECTION('ref_axis',(-1.,0.,1.4081690688991E-16));
#116736=DIRECTION('center_axis',(-1.4081690688991E-16,0.,-1.));
#116737=DIRECTION('ref_axis',(-1.,0.,1.4081690688991E-16));
#116738=DIRECTION('center_axis',(-1.4081690688991E-16,0.,-1.));
#116739=DIRECTION('ref_axis',(-1.,0.,1.4081690688991E-16));
#116740=DIRECTION('',(-0.743144825477393,0.669130606358859,1.04647355694969E-16));
#116741=DIRECTION('center_axis',(1.4081690688991E-16,0.,1.));
#116742=DIRECTION('ref_axis',(1.,0.,-1.4081690688991E-16));
#116743=DIRECTION('',(0.334565226058178,-0.371579467697514,0.866022406579802));
#116744=DIRECTION('center_axis',(1.4081690688991E-16,0.,1.));
#116745=DIRECTION('ref_axis',(-1.,0.,1.40816906889911E-16));
#116746=DIRECTION('',(-0.371579467697534,0.334565226058199,-0.866022406579786));
#116747=DIRECTION('center_axis',(-1.4081690688991E-16,0.,-1.));
#116748=DIRECTION('ref_axis',(-1.,0.,1.40816906889911E-16));
#116749=DIRECTION('center_axis',(-1.4081690688991E-16,0.,-1.));
#116750=DIRECTION('ref_axis',(-1.,0.,1.4081690688991E-16));
#116751=DIRECTION('',(0.669130606358857,-0.743144825477395,-9.42249022928245E-17));
#116752=DIRECTION('center_axis',(1.4081690688991E-16,0.,1.));
#116753=DIRECTION('ref_axis',(-1.,0.,1.4081690688991E-16));
#116754=DIRECTION('',(-0.743144825477393,0.669130606358859,1.04647355694969E-16));
#116755=DIRECTION('center_axis',(-1.4081690688991E-16,0.,-1.));
#116756=DIRECTION('ref_axis',(-1.,0.,1.4081690688991E-16));
#116757=DIRECTION('center_axis',(-1.4081690688991E-16,0.,-1.));
#116758=DIRECTION('ref_axis',(1.,-8.88178419700125E-16,-1.4081690688991E-16));
#116759=DIRECTION('',(0.334572082386297,-0.3715730258176,-0.866022521746663));
#116760=DIRECTION('center_axis',(-1.4081690688991E-16,0.,-1.));
#116761=DIRECTION('ref_axis',(-1.,0.,1.4081690688991E-16));
#116762=DIRECTION('center_axis',(-1.4081690688991E-16,0.,-1.));
#116763=DIRECTION('ref_axis',(-1.,0.,1.4081690688991E-16));
#116764=DIRECTION('center_axis',(-1.4081690688991E-16,0.,-1.));
#116765=DIRECTION('ref_axis',(-1.,0.,1.4081690688991E-16));
#116766=DIRECTION('',(-0.371573025817621,0.334572082386318,0.866022521746647));
#116767=DIRECTION('center_axis',(-1.4081690688991E-16,0.,-1.));
#116768=DIRECTION('ref_axis',(-1.,0.,1.40816906889911E-16));
#116769=DIRECTION('',(0.669130606358857,-0.743144825477395,-9.42249022928245E-17));
#116770=DIRECTION('center_axis',(1.4081690688991E-16,0.,1.));
#116771=DIRECTION('ref_axis',(-1.,-1.06581410364015E-14,1.4081690688991E-16));
#116772=DIRECTION('',(-0.743144825477393,0.669130606358859,1.04647355694969E-16));
#116773=DIRECTION('center_axis',(-1.4081690688991E-16,0.,-1.));
#116774=DIRECTION('ref_axis',(-1.,0.,1.17174841180864E-16));
#116775=DIRECTION('center_axis',(-0.742428258814693,-0.66992557829324,7.86457228688268E-6));
#116776=DIRECTION('ref_axis',(-4.85763185428401E-6,-6.35612262957243E-6,
-0.999999999968002));
#116777=DIRECTION('center_axis',(0.669925578293269,0.742428258814666,7.86457233399125E-6));
#116778=DIRECTION('ref_axis',(-0.629609650280318,0.56813001348582,-0.529924500330469));
#116779=DIRECTION('center_axis',(-1.4081690688991E-16,0.,-1.));
#116780=DIRECTION('ref_axis',(-1.,0.,1.13676889660403E-16));
#116781=DIRECTION('center_axis',(-0.742458811945211,-0.669891716973304,
-9.77059288644529E-6));
#116782=DIRECTION('ref_axis',(0.585911726014151,-0.649388624263268,0.484769908303495));
#116783=DIRECTION('center_axis',(0.669891716943917,0.742458811971727,-9.77052145993168E-6));
#116784=DIRECTION('ref_axis',(0.64939420916695,-0.5859167652342,0.484756336026589));
#116785=DIRECTION('center_axis',(-1.4081690688991E-16,0.,-1.));
#116786=DIRECTION('ref_axis',(-1.,0.,1.15974593313694E-16));
#116787=DIRECTION('center_axis',(0.744880927099454,0.667197425140102,1.81624797774034E-5));
#116788=DIRECTION('ref_axis',(0.577295914342274,-0.644498305797306,-0.501349539850312));
#116789=DIRECTION('center_axis',(-0.667197438400562,-0.744880915222676,
1.81316454311543E-5));
#116790=DIRECTION('ref_axis',(0.645791927483423,-0.578454551166319,-0.498340364241366));
#116791=DIRECTION('center_axis',(-1.4081690688991E-16,0.,-1.));
#116792=DIRECTION('ref_axis',(-1.,0.,1.16261524579732E-16));
#116793=DIRECTION('center_axis',(0.744889942178357,0.667187360266584,1.84940612986181E-5));
#116794=DIRECTION('ref_axis',(0.578432592429571,-0.645812349436537,0.498339387697245));
#116795=DIRECTION('center_axis',(-0.667187373874865,-0.744889929988827,
1.85257057548291E-5));
#116796=DIRECTION('ref_axis',(0.644518813413962,-0.577273915766504,0.501348506860314));
#116797=DIRECTION('center_axis',(-1.4081690688991E-16,0.,-1.));
#116798=DIRECTION('ref_axis',(-1.,0.,1.40816906889911E-16));
#116799=DIRECTION('center_axis',(-1.4081690688991E-16,0.,-1.));
#116800=DIRECTION('ref_axis',(-1.,0.,1.4081690688991E-16));
#116801=DIRECTION('',(0.743144825477393,-0.669130606358859,-1.04647355694969E-16));
#116802=DIRECTION('center_axis',(-1.4081690688991E-16,0.,-1.));
#116803=DIRECTION('ref_axis',(-1.,0.,1.4081690688991E-16));
#116804=DIRECTION('center_axis',(-1.4081690688991E-16,0.,-1.));
#116805=DIRECTION('ref_axis',(-1.,0.,1.4081690688991E-16));
#116806=DIRECTION('center_axis',(-1.4081690688991E-16,0.,-1.));
#116807=DIRECTION('ref_axis',(-1.,0.,1.4081690688991E-16));
#116808=DIRECTION('',(-0.809016994374947,0.587785252292474,1.13923270769252E-16));
#116809=DIRECTION('center_axis',(1.4081690688991E-16,0.,1.));
#116810=DIRECTION('ref_axis',(1.,0.,-1.4081690688991E-16));
#116811=DIRECTION('',(0.371573073483898,-0.334572327551837,0.866022406579805));
#116812=DIRECTION('center_axis',(1.4081690688991E-16,0.,1.));
#116813=DIRECTION('ref_axis',(-1.,0.,1.40816906889911E-16));
#116814=DIRECTION('',(-0.404515505437166,0.293891812003437,-0.86602240657979));
#116815=DIRECTION('center_axis',(-1.4081690688991E-16,0.,-1.));
#116816=DIRECTION('ref_axis',(-1.,0.,1.40816906889911E-16));
#116817=DIRECTION('center_axis',(-1.4081690688991E-16,0.,-1.));
#116818=DIRECTION('ref_axis',(-1.,0.,1.4081690688991E-16));
#116819=DIRECTION('',(0.743144825477393,-0.669130606358859,-1.04647355694969E-16));
#116820=DIRECTION('center_axis',(1.4081690688991E-16,0.,1.));
#116821=DIRECTION('ref_axis',(-1.,0.,1.4081690688991E-16));
#116822=DIRECTION('',(-0.809016994374947,0.587785252292474,1.13923270769252E-16));
#116823=DIRECTION('center_axis',(-1.4081690688991E-16,0.,-1.));
#116824=DIRECTION('ref_axis',(-1.,0.,1.4081690688991E-16));
#116825=DIRECTION('center_axis',(-1.4081690688991E-16,0.,-1.));
#116826=DIRECTION('ref_axis',(1.,0.,-1.4081690688991E-16));
#116827=DIRECTION('',(0.371579218892551,-0.33456520427975,-0.866022521746664));
#116828=DIRECTION('center_axis',(-1.4081690688991E-16,0.,-1.));
#116829=DIRECTION('ref_axis',(-1.,0.,1.4081690688991E-16));
#116830=DIRECTION('center_axis',(-1.4081690688991E-16,0.,-1.));
#116831=DIRECTION('ref_axis',(-1.,0.,1.4081690688991E-16));
#116832=DIRECTION('center_axis',(-1.4081690688991E-16,0.,-1.));
#116833=DIRECTION('ref_axis',(-1.,0.,1.4081690688991E-16));
#116834=DIRECTION('',(-0.404509815527947,0.29389930413172,0.866022521746656));
#116835=DIRECTION('center_axis',(-1.4081690688991E-16,0.,-1.));
#116836=DIRECTION('ref_axis',(-1.,0.,1.40816906889911E-16));
#116837=DIRECTION('',(0.743144825477393,-0.669130606358859,-1.04647355694969E-16));
#116838=DIRECTION('center_axis',(1.4081690688991E-16,0.,1.));
#116839=DIRECTION('ref_axis',(-1.,-1.06581410364015E-14,1.4081690688991E-16));
#116840=DIRECTION('',(-0.809016994374947,0.587785252292474,1.13923270769252E-16));
#116841=DIRECTION('center_axis',(-1.4081690688991E-16,0.,-1.));
#116842=DIRECTION('ref_axis',(-1.,0.,1.17174841180864E-16));
#116843=DIRECTION('center_axis',(-0.668334867928773,-0.743860540860166,
7.86457209247282E-6));
#116844=DIRECTION('ref_axis',(-4.16662536933619E-6,-6.82906378195756E-6,
-0.999999999968002));
#116845=DIRECTION('center_axis',(0.58865077089958,0.808387450333983,7.86457252685304E-6));
#116846=DIRECTION('ref_axis',(-0.685546339984752,0.499205608625359,-0.529924500330467));
#116847=DIRECTION('center_axis',(-1.4081690688991E-16,0.,-1.));
#116848=DIRECTION('ref_axis',(-1.,0.,1.13676889660403E-16));
#116849=DIRECTION('center_axis',(-0.668368793160425,-0.74383005870549,-9.77058632101317E-6));
#116850=DIRECTION('ref_axis',(0.650581635232264,-0.5845867531026,0.484769908302354));
#116851=DIRECTION('center_axis',(0.588613901374041,0.808414296641126,-9.77052680656433E-6));
#116852=DIRECTION('ref_axis',(0.707081738813996,-0.514826873149213,0.484756336027885));
#116853=DIRECTION('center_axis',(-1.4081690688991E-16,0.,-1.));
#116854=DIRECTION('ref_axis',(-1.,0.,1.15974593313694E-16));
#116855=DIRECTION('center_axis',(0.671059269896534,0.741403706462312,1.81624796124116E-5));
#116856=DIRECTION('ref_axis',(0.641501844408008,-0.580623821870257,-0.50134953984012));
#116857=DIRECTION('center_axis',(-0.585681203637444,-0.81054150256297,1.8131645301284E-5));
#116858=DIRECTION('ref_axis',(0.702719177032194,-0.50778207883572,-0.49834036425366));
#116859=DIRECTION('center_axis',(-1.4081690688991E-16,0.,-1.));
#116860=DIRECTION('ref_axis',(-1.,0.,1.16261524579732E-16));
#116861=DIRECTION('center_axis',(0.671069287652099,0.741394639060787,1.84940697053889E-5));
#116862=DIRECTION('ref_axis',(0.642769650611578,-0.581811851823098,0.498339387697629));
#116863=DIRECTION('center_axis',(-0.585670251953324,-0.81054941591104,1.85257201982103E-5));
#116864=DIRECTION('ref_axis',(0.701329627214891,-0.50674098774034,0.501348506863805));
#116865=DIRECTION('center_axis',(-1.4081690688991E-16,0.,-1.));
#116866=DIRECTION('ref_axis',(-1.,0.,1.40816906889911E-16));
#116867=DIRECTION('center_axis',(-1.4081690688991E-16,0.,-1.));
#116868=DIRECTION('ref_axis',(-1.,0.,1.4081690688991E-16));
#116869=DIRECTION('',(0.809016994374947,-0.587785252292474,-1.13923270769252E-16));
#116870=DIRECTION('center_axis',(-1.4081690688991E-16,0.,-1.));
#116871=DIRECTION('ref_axis',(-1.,0.,1.4081690688991E-16));
#116872=DIRECTION('center_axis',(-1.4081690688991E-16,0.,-1.));
#116873=DIRECTION('ref_axis',(-1.,0.,1.4081690688991E-16));
#116874=DIRECTION('center_axis',(-1.4081690688991E-16,0.,-1.));
#116875=DIRECTION('ref_axis',(-1.,0.,1.4081690688991E-16));
#116876=DIRECTION('',(-0.866025403784438,0.500000000000001,1.2195101864901E-16));
#116877=DIRECTION('center_axis',(1.4081690688991E-16,0.,1.));
#116878=DIRECTION('ref_axis',(1.,0.,-1.4081690688991E-16));
#116879=DIRECTION('',(0.404509888559909,-0.293899542971724,0.866022406579796));
#116880=DIRECTION('center_axis',(1.4081690688991E-16,0.,1.));
#116881=DIRECTION('ref_axis',(-1.,0.,1.40816906889911E-16));
#116882=DIRECTION('',(-0.433019586648901,0.249998457755605,-0.86602240657978));
#116883=DIRECTION('center_axis',(-1.4081690688991E-16,0.,-1.));
#116884=DIRECTION('ref_axis',(-1.,0.,1.40816906889911E-16));
#116885=DIRECTION('center_axis',(-1.4081690688991E-16,0.,-1.));
#116886=DIRECTION('ref_axis',(-1.,0.,1.4081690688991E-16));
#116887=DIRECTION('',(0.809016994374947,-0.587785252292474,-1.13923270769252E-16));
#116888=DIRECTION('center_axis',(1.4081690688991E-16,0.,1.));
#116889=DIRECTION('ref_axis',(-1.,0.,1.4081690688991E-16));
#116890=DIRECTION('',(-0.866025403784438,0.500000000000001,1.2195101864901E-16));
#116891=DIRECTION('center_axis',(-1.4081690688991E-16,0.,-1.));
#116892=DIRECTION('ref_axis',(-1.,0.,1.4081690688991E-16));
#116893=DIRECTION('center_axis',(-1.4081690688991E-16,0.,-1.));
#116894=DIRECTION('ref_axis',(1.,0.,-1.4081690688991E-16));
#116895=DIRECTION('',(0.40451525571868,-0.293891816351526,-0.866022521746664));
#116896=DIRECTION('center_axis',(-1.4081690688991E-16,0.,-1.));
#116897=DIRECTION('ref_axis',(-1.,0.,1.4081690688991E-16));
#116898=DIRECTION('center_axis',(-1.4081690688991E-16,0.,-1.));
#116899=DIRECTION('ref_axis',(-1.,0.,1.4081690688991E-16));
#116900=DIRECTION('center_axis',(-1.4081690688991E-16,0.,-1.));
#116901=DIRECTION('ref_axis',(-1.,0.,1.4081690688991E-16));
#116902=DIRECTION('',(-0.433014711050233,0.250006503598672,0.866022521746663));
#116903=DIRECTION('center_axis',(-1.4081690688991E-16,0.,-1.));
#116904=DIRECTION('ref_axis',(-1.,0.,1.40816906889911E-16));
#116905=DIRECTION('',(0.809016994374947,-0.587785252292474,-1.13923270769252E-16));
#116906=DIRECTION('center_axis',(1.4081690688991E-16,0.,1.));
#116907=DIRECTION('ref_axis',(-1.,-1.24344978758018E-14,1.4081690688991E-16));
#116908=DIRECTION('',(-0.866025403784438,0.500000000000001,1.2195101864901E-16));
#116909=DIRECTION('center_axis',(-1.4081690688991E-16,0.,-1.));
#116910=DIRECTION('ref_axis',(-1.,0.,1.17174841180864E-16));
#116911=DIRECTION('center_axis',(-0.586919060371807,-0.809645611678606,
7.86457181291275E-6));
#116912=DIRECTION('ref_axis',(-3.4299684348052E-6,-7.2271841840149E-6,-0.999999999968002));
#116913=DIRECTION('center_axis',(0.500926582476729,0.86548977978156,7.86457235433928E-6));
#116914=DIRECTION('ref_axis',(-0.733972040528699,0.424811802651075,-0.529924500330455));
#116915=DIRECTION('center_axis',(-1.4081690688991E-16,0.,-1.));
#116916=DIRECTION('ref_axis',(-1.,0.,1.13676889660403E-16));
#116917=DIRECTION('center_axis',(-0.586955986008474,-0.809618842662,-9.77058993673793E-6));
#116918=DIRECTION('ref_axis',(0.708123635911361,-0.513380027141697,0.484769908302552));
#116919=DIRECTION('center_axis',(0.500887108719152,0.86551262510925,-9.77051851264757E-6));
#116920=DIRECTION('ref_axis',(0.757022332965959,-0.438096430108722,0.484756336025401));
#116921=DIRECTION('center_axis',(-1.4081690688991E-16,0.,-1.));
#116922=DIRECTION('ref_axis',(-1.,0.,1.15974593313694E-16));
#116923=DIRECTION('center_axis',(0.589885346904599,0.80748701362769,1.81624796986456E-5));
#116924=DIRECTION('ref_axis',(0.698679346015346,-0.510387901840021,-0.501349539849106));
#116925=DIRECTION('center_axis',(-0.497748123045557,-0.867321627584524,
1.81316453122383E-5));
#116926=DIRECTION('ref_axis',(0.751947288228285,-0.431546239793356,-0.498340364255539));
#116927=DIRECTION('center_axis',(-1.4081690688991E-16,0.,-1.));
#116928=DIRECTION('ref_axis',(-1.,0.,1.16261524579732E-16));
#116929=DIRECTION('center_axis',(0.589896257578203,0.807479043042728,1.84940806699832E-5));
#116930=DIRECTION('ref_axis',(0.700064389992645,-0.511436901808749,0.498339387699282));
#116931=DIRECTION('center_axis',(-0.497736404182369,-0.8673283528217,1.85257135242689E-5));
#116932=DIRECTION('ref_axis',(0.750456526858729,-0.430656099411321,0.501348506864197));
#116933=DIRECTION('center_axis',(-1.4081690688991E-16,0.,-1.));
#116934=DIRECTION('ref_axis',(-1.,0.,1.40816906889911E-16));
#116935=DIRECTION('center_axis',(-1.4081690688991E-16,0.,-1.));
#116936=DIRECTION('ref_axis',(-1.,0.,1.4081690688991E-16));
#116937=DIRECTION('',(0.866025403784438,-0.500000000000001,-1.2195101864901E-16));
#116938=DIRECTION('center_axis',(-1.4081690688991E-16,0.,-1.));
#116939=DIRECTION('ref_axis',(-1.,0.,1.4081690688991E-16));
#116940=DIRECTION('center_axis',(-1.4081690688991E-16,0.,-1.));
#116941=DIRECTION('ref_axis',(-1.,0.,1.4081690688991E-16));
#116942=DIRECTION('center_axis',(-1.4081690688991E-16,0.,-1.));
#116943=DIRECTION('ref_axis',(-1.,0.,1.4081690688991E-16));
#116944=DIRECTION('',(-0.913545457642601,0.406736643075801,1.28642645648559E-16));
#116945=DIRECTION('center_axis',(1.4081690688991E-16,0.,1.));
#116946=DIRECTION('ref_axis',(1.,0.,-1.4081690688991E-16));
#116947=DIRECTION('',(0.433014808647712,-0.250006733496369,0.866022406579795));
#116948=DIRECTION('center_axis',(1.4081690688991E-16,0.,1.));
#116949=DIRECTION('ref_axis',(-1.,0.,1.40816906889911E-16));
#116950=DIRECTION('',(-0.456779414654131,0.203366068089033,-0.866022406579781));
#116951=DIRECTION('center_axis',(-1.4081690688991E-16,0.,-1.));
#116952=DIRECTION('ref_axis',(-1.,0.,1.40816906889911E-16));
#116953=DIRECTION('center_axis',(-1.4081690688991E-16,0.,-1.));
#116954=DIRECTION('ref_axis',(-1.,0.,1.4081690688991E-16));
#116955=DIRECTION('',(0.866025403784438,-0.500000000000001,-1.2195101864901E-16));
#116956=DIRECTION('center_axis',(1.4081690688991E-16,0.,1.));
#116957=DIRECTION('ref_axis',(-1.,1.24344978758018E-14,1.4081690688991E-16));
#116958=DIRECTION('',(-0.913545457642601,0.406736643075801,1.28642645648559E-16));
#116959=DIRECTION('center_axis',(-1.4081690688991E-16,0.,-1.));
#116960=DIRECTION('ref_axis',(-1.,0.,1.4081690688991E-16));
#116961=DIRECTION('center_axis',(-1.4081690688991E-16,0.,-1.));
#116962=DIRECTION('ref_axis',(1.,0.,-1.4081690688991E-16));
#116963=DIRECTION('',(0.433019338752905,-0.249998488182556,-0.866022521746654));
#116964=DIRECTION('center_axis',(-1.4081690688991E-16,0.,-1.));
#116965=DIRECTION('ref_axis',(-1.,0.,1.4081690688991E-16));
#116966=DIRECTION('center_axis',(-1.4081690688991E-16,0.,-1.));
#116967=DIRECTION('ref_axis',(-1.,0.,1.4081690688991E-16));
#116968=DIRECTION('center_axis',(-1.4081690688991E-16,0.,-1.));
#116969=DIRECTION('ref_axis',(-1.,0.,1.4081690688991E-16));
#116970=DIRECTION('',(-0.456775406784136,0.203374579494979,0.86602252174665));
#116971=DIRECTION('center_axis',(-1.4081690688991E-16,0.,-1.));
#116972=DIRECTION('ref_axis',(-1.,0.,1.40816906889911E-16));
#116973=DIRECTION('',(0.866025403784438,-0.500000000000001,-1.2195101864901E-16));
#116974=DIRECTION('center_axis',(1.4081690688991E-16,0.,1.));
#116975=DIRECTION('ref_axis',(-1.,0.,1.4081690688991E-16));
#116976=DIRECTION('',(-0.913545457642601,0.406736643075801,1.28642645648559E-16));
#116977=DIRECTION('center_axis',(-1.4081690688991E-16,0.,-1.));
#116978=DIRECTION('ref_axis',(-1.,0.,1.17174841180864E-16));
#116979=DIRECTION('center_axis',(-0.499072844768411,-0.866560035746465,
7.86457214289953E-6));
#116980=DIRECTION('ref_axis',(-2.655732390574E-6,-7.54612254363985E-6,-0.999999999968002));
#116981=DIRECTION('center_axis',(0.407714137590715,0.913109622086422,7.86457249655275E-6));
#116982=DIRECTION('ref_axis',(-0.774356189802951,0.345763669669564,-0.529924500330464));
#116983=DIRECTION('center_axis',(-1.4081690688991E-16,0.,-1.));
#116984=DIRECTION('ref_axis',(-1.,0.,1.13676889660403E-16));
#116985=DIRECTION('center_axis',(-0.499112366248818,-0.866537273152195,
-9.77058602131441E-6));
#116986=DIRECTION('ref_axis',(0.757907285848944,-0.43654860217067,0.484769908306942));
#116987=DIRECTION('center_axis',(0.407672492086804,0.913128216134116,-9.77051719973362E-6));
#116988=DIRECTION('ref_axis',(0.798668832020144,-0.356566110901745,0.484756336024588));
#116989=DIRECTION('center_axis',(-1.4081690688991E-16,0.,-1.));
#116990=DIRECTION('ref_axis',(-1.,0.,1.15974593313694E-16));
#116991=DIRECTION('center_axis',(0.502248516610394,0.864723324094351,1.81624796546292E-5));
#116992=DIRECTION('ref_axis',(0.748201970509818,-0.434560065158728,-0.501349539836697));
#116993=DIRECTION('center_axis',(-0.404361609857007,-0.91459919535559,1.81316453037353E-5));
#116994=DIRECTION('ref_axis',(0.792936907584003,-0.350582289843111,-0.498340364248652));
#116995=DIRECTION('center_axis',(-1.4081690688991E-16,0.,-1.));
#116996=DIRECTION('ref_axis',(-1.,0.,1.16261524579732E-16));
#116997=DIRECTION('center_axis',(0.502260200679148,0.864716537642083,1.84940567917327E-5));
#116998=DIRECTION('ref_axis',(0.74968907742121,-0.435458542074672,0.498339387696313));
#116999=DIRECTION('center_axis',(-0.404349252215734,-0.914604658794921,
1.85257199402894E-5));
#117000=DIRECTION('ref_axis',(0.791361267754418,-0.349852852738104,0.501348506858384));
#117001=DIRECTION('center_axis',(-1.4081690688991E-16,0.,-1.));
#117002=DIRECTION('ref_axis',(-1.,0.,1.40816906889911E-16));
#117003=DIRECTION('center_axis',(-1.4081690688991E-16,0.,-1.));
#117004=DIRECTION('ref_axis',(-1.,0.,1.4081690688991E-16));
#117005=DIRECTION('',(0.913545457642601,-0.406736643075801,-1.28642645648559E-16));
#117006=DIRECTION('center_axis',(-1.4081690688991E-16,0.,-1.));
#117007=DIRECTION('ref_axis',(-1.,0.,1.4081690688991E-16));
#117008=DIRECTION('center_axis',(-1.4081690688991E-16,0.,-1.));
#117009=DIRECTION('ref_axis',(-1.,0.,1.4081690688991E-16));
#117010=DIRECTION('center_axis',(-1.4081690688991E-16,0.,-1.));
#117011=DIRECTION('ref_axis',(-1.,0.,1.4081690688991E-16));
#117012=DIRECTION('',(-0.951056516295153,0.309016994374948,1.33924836902177E-16));
#117013=DIRECTION('center_axis',(1.4081690688991E-16,0.,1.));
#117014=DIRECTION('ref_axis',(1.,0.,-1.4081690688991E-16));
#117015=DIRECTION('',(0.456775527877821,-0.203374797931565,0.86602240657978));
#117016=DIRECTION('center_axis',(1.4081690688991E-16,0.,1.));
#117017=DIRECTION('ref_axis',(-1.,0.,1.40816906889911E-16));
#117018=DIRECTION('',(-0.475534671805141,0.15450555722341,-0.866022406579795));
#117019=DIRECTION('center_axis',(-1.4081690688991E-16,0.,-1.));
#117020=DIRECTION('ref_axis',(-1.,0.,1.40816906889911E-16));
#117021=DIRECTION('center_axis',(-1.4081690688991E-16,0.,-1.));
#117022=DIRECTION('ref_axis',(-1.,0.,1.4081690688991E-16));
#117023=DIRECTION('',(0.9135454576426,-0.406736643075801,-1.28642645648559E-16));
#117024=DIRECTION('center_axis',(1.4081690688991E-16,0.,1.));
#117025=DIRECTION('ref_axis',(-1.,-1.24344978758018E-14,1.4081690688991E-16));
#117026=DIRECTION('',(-0.951056516295153,0.309016994374948,1.33924836902177E-16));
#117027=DIRECTION('center_axis',(-1.4081690688991E-16,0.,-1.));
#117028=DIRECTION('ref_axis',(-1.,0.,1.4081690688991E-16));
#117029=DIRECTION('center_axis',(-1.4081690688991E-16,0.,-1.));
#117030=DIRECTION('ref_axis',(1.,0.,-1.4081690688991E-16));
#117031=DIRECTION('',(0.456779171296642,-0.203366124261506,-0.866022521746638));
#117032=DIRECTION('center_axis',(-1.4081690688991E-16,0.,-1.));
#117033=DIRECTION('ref_axis',(-1.,0.,1.4081690688991E-16));
#117034=DIRECTION('center_axis',(-1.4081690688991E-16,0.,-1.));
#117035=DIRECTION('ref_axis',(-1.,0.,1.4081690688991E-16));
#117036=DIRECTION('center_axis',(-1.4081690688991E-16,0.,-1.));
#117037=DIRECTION('ref_axis',(-1.,0.,1.4081690688991E-16));
#117038=DIRECTION('',(-0.47553157557488,0.154514440939486,0.866022521746652));
#117039=DIRECTION('center_axis',(-1.4081690688991E-16,0.,-1.));
#117040=DIRECTION('ref_axis',(-1.,0.,1.40816906889911E-16));
#117041=DIRECTION('',(0.913545457642601,-0.406736643075801,-1.28642645648559E-16));
#117042=DIRECTION('center_axis',(1.4081690688991E-16,0.,1.));
#117043=DIRECTION('ref_axis',(-1.,-1.24344978758018E-14,1.4081690688991E-16));
#117044=DIRECTION('',(-0.951056516295153,0.309016994374948,1.33924836902177E-16));
#117045=DIRECTION('center_axis',(-1.4081690688991E-16,0.,-1.));
#117046=DIRECTION('ref_axis',(-1.,0.,1.17174841180864E-16));
#117047=DIRECTION('center_axis',(-0.405758682640351,-0.913980246723153,
7.86457178216999E-6));
#117048=DIRECTION('ref_axis',(-1.85239931600463E-6,-7.78238337918387E-6,
-0.999999999968002));
#117049=DIRECTION('center_axis',(0.310034691293422,0.950725244291294,7.86457224375456E-6));
#117050=DIRECTION('ref_axis',(-0.806256330617395,0.262927277567121,-0.529924500330488));
#117051=DIRECTION('center_axis',(-1.4081690688991E-16,0.,-1.));
#117052=DIRECTION('ref_axis',(-1.,0.,1.13676889660403E-16));
#117053=DIRECTION('center_axis',(-0.405800366957686,-0.913961739944043,
-9.77058414968768E-6));
#117054=DIRECTION('ref_axis',(0.799387144964551,-0.354934259362886,0.48476990830284));
#117055=DIRECTION('center_axis',(0.309991330319367,0.95073938333876,-9.77051439570099E-6));
#117056=DIRECTION('ref_axis',(0.831564948216299,-0.271129178766668,0.484756336028046));
#117057=DIRECTION('center_axis',(-1.4081690688991E-16,0.,-1.));
#117058=DIRECTION('ref_axis',(-1.,0.,1.15974593313694E-16));
#117059=DIRECTION('center_axis',(0.409108946466091,0.912485544867166,1.81624799040554E-5));
#117060=DIRECTION('ref_axis',(0.789527137636282,-0.353971097460886,-0.501349539840415));
#117061=DIRECTION('center_axis',(-0.306544826252881,-0.951856222950102,
1.81316451570291E-5));
#117062=DIRECTION('ref_axis',(0.825238944244478,-0.265777286959491,-0.498340364247882));
#117063=DIRECTION('center_axis',(-1.4081690688991E-16,0.,-1.));
#117064=DIRECTION('ref_axis',(-1.,0.,1.16261524579732E-16));
#117065=DIRECTION('center_axis',(0.40912127591188,0.912480016906785,1.84940449550723E-5));
#117066=DIRECTION('ref_axis',(0.791100014435804,-0.354709207428031,0.498339387692211));
#117067=DIRECTION('center_axis',(-0.306531965214468,-0.951860364737683,
1.85257042376944E-5));
#117068=DIRECTION('ref_axis',(0.823595688991461,-0.265216544996207,0.501348506864193));
#117069=DIRECTION('center_axis',(-1.4081690688991E-16,0.,-1.));
#117070=DIRECTION('ref_axis',(-1.,0.,1.40816906889911E-16));
#117071=DIRECTION('center_axis',(-1.4081690688991E-16,0.,-1.));
#117072=DIRECTION('ref_axis',(-1.,0.,1.4081690688991E-16));
#117073=DIRECTION('',(0.951056516295153,-0.309016994374948,-1.33924836902177E-16));
#117074=DIRECTION('center_axis',(-1.4081690688991E-16,0.,-1.));
#117075=DIRECTION('ref_axis',(-1.,0.,1.4081690688991E-16));
#117076=DIRECTION('center_axis',(-1.4081690688991E-16,0.,-1.));
#117077=DIRECTION('ref_axis',(-1.,0.,1.4081690688991E-16));
#117078=DIRECTION('center_axis',(-1.4081690688991E-16,0.,-1.));
#117079=DIRECTION('ref_axis',(-1.,0.,1.4081690688991E-16));
#117080=DIRECTION('',(-0.978147600733806,0.20791169081776,1.37739719617122E-16));
#117081=DIRECTION('center_axis',(1.4081690688991E-16,0.,1.));
#117082=DIRECTION('ref_axis',(1.,0.,-1.4081690688991E-16));
#117083=DIRECTION('',(0.475531718838045,-0.154514645521707,0.866022406579781));
#117084=DIRECTION('center_axis',(1.4081690688991E-16,0.,1.));
#117085=DIRECTION('ref_axis',(-1.,0.,1.40816906889911E-16));
#117086=DIRECTION('',(-0.489079871579872,0.103952251140493,-0.866022406579784));
#117087=DIRECTION('center_axis',(-1.4081690688991E-16,0.,-1.));
#117088=DIRECTION('ref_axis',(-1.,0.,1.40816906889911E-16));
#117089=DIRECTION('center_axis',(-1.4081690688991E-16,0.,-1.));
#117090=DIRECTION('ref_axis',(-1.,0.,1.4081690688991E-16));
#117091=DIRECTION('',(0.951056516295153,-0.309016994374948,-1.33924836902177E-16));
#117092=DIRECTION('center_axis',(1.4081690688991E-16,0.,1.));
#117093=DIRECTION('ref_axis',(-1.,0.,1.4081690688991E-16));
#117094=DIRECTION('',(-0.978147600733806,0.20791169081776,1.37739719617122E-16));
#117095=DIRECTION('center_axis',(-1.4081690688991E-16,0.,-1.));
#117096=DIRECTION('ref_axis',(-1.,0.,1.4081690688991E-16));
#117097=DIRECTION('center_axis',(-1.4081690688991E-16,0.,-1.));
#117098=DIRECTION('ref_axis',(1.,0.,-1.4081690688991E-16));
#117099=DIRECTION('',(0.475534435652401,-0.154505638525951,-0.866022521746658));
#117100=DIRECTION('center_axis',(-1.4081690688991E-16,0.,-1.));
#117101=DIRECTION('ref_axis',(-1.,0.,1.4081690688991E-16));
#117102=DIRECTION('center_axis',(-1.4081690688991E-16,0.,-1.));
#117103=DIRECTION('ref_axis',(-1.,0.,1.4081690688991E-16));
#117104=DIRECTION('center_axis',(-1.4081690688991E-16,0.,-1.));
#117105=DIRECTION('ref_axis',(-1.,0.,1.4081690688991E-16));
#117106=DIRECTION('',(-0.489077720912242,0.103961409834797,0.866022521746662));
#117107=DIRECTION('center_axis',(-1.4081690688991E-16,0.,-1.));
#117108=DIRECTION('ref_axis',(-1.,0.,1.40816906889911E-16));
#117109=DIRECTION('',(0.951056516295153,-0.309016994374948,-1.33924836902177E-16));
#117110=DIRECTION('center_axis',(1.4081690688991E-16,0.,1.));
#117111=DIRECTION('ref_axis',(-1.,-1.33226762955019E-14,1.4081690688991E-16));
#117112=DIRECTION('',(-0.978147600733806,0.20791169081776,1.37739719617122E-16));
#117113=DIRECTION('center_axis',(-1.4081690688991E-16,0.,-1.));
#117114=DIRECTION('ref_axis',(-1.,0.,1.17174841180864E-16));
#117115=DIRECTION('center_axis',(-0.307998943474356,-0.951386698854272,
7.86457226542829E-6));
#117116=DIRECTION('ref_axis',(-1.0287712269461E-6,-7.93337958510981E-6,
-0.999999999968001));
#117117=DIRECTION('center_axis',(0.208958440039612,0.977924521767585,7.86457233133809E-6));
#117118=DIRECTION('ref_axis',(-0.829322958353501,0.177210199190947,-0.529924500330474));
#117119=DIRECTION('center_axis',(-1.4081690688991E-16,0.,-1.));
#117120=DIRECTION('ref_axis',(-1.,0.,1.13676889660403E-16));
#117121=DIRECTION('center_axis',(-0.308042333923157,-0.95137265065573,-9.77058986043835E-6));
#117122=DIRECTION('ref_axis',(0.83210875123643,-0.269431182534026,0.484769908300902));
#117123=DIRECTION('center_axis',(0.208913838670723,0.977934050903434,-9.77051847801327E-6));
#117124=DIRECTION('ref_axis',(0.855350264825764,-0.182721698612452,0.484756336027365));
#117125=DIRECTION('center_axis',(-1.4081690688991E-16,0.,-1.));
#117126=DIRECTION('ref_axis',(-1.,0.,1.15974593313694E-16));
#117127=DIRECTION('center_axis',(0.311487093092649,0.950250383060599,1.81624798352045E-5));
#117128=DIRECTION('ref_axis',(0.822202080223852,-0.269503948346651,-0.501349539843347));
#117129=DIRECTION('center_axis',(-0.20536947338361,-0.978684514577288,1.81316452437622E-5));
#117130=DIRECTION('ref_axis',(0.848499490336976,-0.178060372501888,-0.498340364251564));
#117131=DIRECTION('center_axis',(-1.4081690688991E-16,0.,-1.));
#117132=DIRECTION('ref_axis',(-1.,0.,1.16261524579732E-16));
#117133=DIRECTION('center_axis',(0.311499932820754,0.950246174162588,1.84940539067784E-5));
#117134=DIRECTION('ref_axis',(0.8238434941389,-0.270073604474909,0.49833938769772));
#117135=DIRECTION('center_axis',(-0.205356249870299,-0.97868728932995,1.85257143532325E-5));
#117136=DIRECTION('ref_axis',(0.846806623515352,-0.177674469288616,0.501348506862778));
#117137=DIRECTION('center_axis',(-1.4081690688991E-16,0.,-1.));
#117138=DIRECTION('ref_axis',(-1.,0.,1.40816906889911E-16));
#117139=DIRECTION('center_axis',(-1.4081690688991E-16,0.,-1.));
#117140=DIRECTION('ref_axis',(-1.,0.,1.4081690688991E-16));
#117141=DIRECTION('',(0.978147600733806,-0.20791169081776,-1.37739719617122E-16));
#117142=DIRECTION('center_axis',(-1.4081690688991E-16,0.,-1.));
#117143=DIRECTION('ref_axis',(-1.,0.,1.4081690688991E-16));
#117144=DIRECTION('center_axis',(-1.4081690688991E-16,0.,-1.));
#117145=DIRECTION('ref_axis',(-1.,0.,1.4081690688991E-16));
#117146=DIRECTION('center_axis',(-1.4081690688991E-16,0.,-1.));
#117147=DIRECTION('ref_axis',(-1.,0.,1.4081690688991E-16));
#117148=DIRECTION('',(-0.994521895368273,0.104528463267654,1.40045497140051E-16));
#117149=DIRECTION('center_axis',(1.4081690688991E-16,0.,1.));
#117150=DIRECTION('ref_axis',(1.,0.,-1.4081690688991E-16));
#117151=DIRECTION('',(0.489077884775266,-0.103961598321233,0.866022406579787));
#117152=DIRECTION('center_axis',(1.4081690688991E-16,0.,1.));
#117153=DIRECTION('ref_axis',(-1.,0.,1.40816906889911E-16));
#117154=DIRECTION('',(-0.497266609935056,0.0522600224406417,-0.866022406579761));
#117155=DIRECTION('center_axis',(-1.4081690688991E-16,0.,-1.));
#117156=DIRECTION('ref_axis',(-1.,0.,1.40816906889911E-16));
#117157=DIRECTION('center_axis',(-1.4081690688991E-16,0.,-1.));
#117158=DIRECTION('ref_axis',(-1.,0.,1.4081690688991E-16));
#117159=DIRECTION('',(0.978147600733806,-0.20791169081776,-1.37739719617122E-16));
#117160=DIRECTION('center_axis',(1.4081690688991E-16,0.,1.));
#117161=DIRECTION('ref_axis',(-1.,0.,1.4081690688991E-16));
#117162=DIRECTION('',(-0.994521895368273,0.104528463267654,1.40045497140051E-16));
#117163=DIRECTION('center_axis',(-1.4081690688991E-16,0.,-1.));
#117164=DIRECTION('ref_axis',(-1.,0.,1.4081690688991E-16));
#117165=DIRECTION('center_axis',(-1.4081690688991E-16,0.,-1.));
#117166=DIRECTION('ref_axis',(1.,0.,-1.4081690688991E-16));
#117167=DIRECTION('',(0.489079645219224,-0.103952356682314,-0.866022521746652));
#117168=DIRECTION('center_axis',(-1.4081690688991E-16,0.,-1.));
#117169=DIRECTION('ref_axis',(-1.,0.,1.4081690688991E-16));
#117170=DIRECTION('center_axis',(-1.4081690688991E-16,0.,-1.));
#117171=DIRECTION('ref_axis',(-1.,0.,1.4081690688991E-16));
#117172=DIRECTION('center_axis',(-1.4081690688991E-16,0.,-1.));
#117173=DIRECTION('ref_axis',(-1.,0.,1.4081690688991E-16));
#117174=DIRECTION('',(-0.497265428393217,0.0522693557686608,0.866022521746657));
#117175=DIRECTION('center_axis',(-1.4081690688991E-16,0.,-1.));
#117176=DIRECTION('ref_axis',(-1.,0.,1.40816906889911E-16));
#117177=DIRECTION('',(0.978147600733806,-0.20791169081776,-1.37739719617122E-16));
#117178=DIRECTION('center_axis',(1.4081690688991E-16,0.,1.));
#117179=DIRECTION('ref_axis',(-1.,0.,1.4081690688991E-16));
#117180=DIRECTION('',(-0.994521895368273,0.104528463267654,1.40045497140051E-16));
#117181=DIRECTION('center_axis',(-1.4081690688991E-16,0.,-1.));
#117182=DIRECTION('ref_axis',(-1.,0.,1.17174841180864E-16));
#117183=DIRECTION('center_axis',(-0.206864703431192,-0.978369559222114,
7.86457194672106E-6));
#117184=DIRECTION('ref_axis',(-1.93871468046092E-7,-7.99745526561114E-6,
-0.999999999968002));
#117185=DIRECTION('center_axis',(0.105592796389255,0.99440945353956,7.86457230629007E-6));
#117186=DIRECTION('ref_axis',(-0.843303350210935,0.0895515687886684,-0.529924500330473));
#117187=DIRECTION('center_axis',(-1.4081690688991E-16,0.,-1.));
#117188=DIRECTION('ref_axis',(-1.,0.,1.13676889660403E-16));
#117189=DIRECTION('center_axis',(-0.206909324622115,-0.978360123517387,
-9.77058412670988E-6));
#117190=DIRECTION('ref_axis',(0.855713599896876,-0.180976161286326,0.484769908304544));
#117191=DIRECTION('center_axis',(0.105547443284639,0.994414268361337,-9.77051707379648E-6));
#117192=DIRECTION('ref_axis',(0.869764184940883,-0.092312281291246,0.484756336025561));
#117193=DIRECTION('center_axis',(-1.4081690688991E-16,0.,-1.));
#117194=DIRECTION('ref_axis',(-1.,0.,1.15974593313694E-16));
#117195=DIRECTION('center_axis',(0.210452521944388,0.977604079204548,1.81624797328856E-5));
#117196=DIRECTION('ref_axis',(0.845868804765148,-0.182084057577678,-0.50134953984344));
#117197=DIRECTION('center_axis',(-0.101944049587622,-0.994790133859861,
1.81316452425136E-5));
#117198=DIRECTION('ref_axis',(0.862463698451802,-0.0883925913418604,-0.498340364257914));
#117199=DIRECTION('center_axis',(-1.4081690688991E-16,0.,-1.));
#117200=DIRECTION('ref_axis',(-1.,0.,1.16261524579732E-16));
#117201=DIRECTION('center_axis',(0.210465731284082,0.977601235480513,1.84940551537643E-5));
#117202=DIRECTION('ref_axis',(0.847560772122061,-0.182479018595766,0.498339387698967));
#117203=DIRECTION('center_axis',(-0.101930608472471,-0.994791511178714,
1.8525712556693E-5));
#117204=DIRECTION('ref_axis',(0.860739767465021,-0.0881857549145027,0.50134850686366));
#117205=DIRECTION('center_axis',(-1.4081690688991E-16,0.,-1.));
#117206=DIRECTION('ref_axis',(-1.,0.,1.40816906889911E-16));
#117207=DIRECTION('center_axis',(-1.4081690688991E-16,0.,-1.));
#117208=DIRECTION('ref_axis',(-1.,0.,1.40816906889911E-16));
#117209=DIRECTION('center_axis',(-1.4081690688991E-16,0.,-1.));
#117210=DIRECTION('ref_axis',(-1.,0.,1.4081690688991E-16));
#117211=DIRECTION('',(0.994521895368273,-0.104528463267654,-1.40045497140051E-16));
#117212=DIRECTION('center_axis',(-1.4081690688991E-16,0.,-1.));
#117213=DIRECTION('ref_axis',(-1.,0.,1.4081690688991E-16));
#117214=DIRECTION('center_axis',(-1.4081690688991E-16,0.,-1.));
#117215=DIRECTION('ref_axis',(-1.,0.,1.4081690688991E-16));
#117216=DIRECTION('center_axis',(-1.4081690688991E-16,0.,-1.));
#117217=DIRECTION('ref_axis',(-1.,0.,1.4081690688991E-16));
#117218=DIRECTION('',(-1.,0.,1.40816906889911E-16));
#117219=DIRECTION('center_axis',(1.4081690688991E-16,0.,1.));
#117220=DIRECTION('ref_axis',(1.,0.,-1.4081690688991E-16));
#117221=DIRECTION('',(0.497265611060779,-0.052269526094198,0.866022406579782));
#117222=DIRECTION('center_axis',(1.4081690688991E-16,0.,1.));
#117223=DIRECTION('ref_axis',(-1.,0.,1.40816906889911E-16));
#117224=DIRECTION('',(-0.500005191251964,-4.77800116594404E-6,-0.866022406579794));
#117225=DIRECTION('center_axis',(-1.4081690688991E-16,0.,-1.));
#117226=DIRECTION('ref_axis',(-1.,0.,1.40816906889911E-16));
#117227=DIRECTION('center_axis',(-1.4081690688991E-16,0.,-1.));
#117228=DIRECTION('ref_axis',(-1.,0.,1.4081690688991E-16));
#117229=DIRECTION('',(0.994521895368273,-0.104528463267654,-1.40045497140051E-16));
#117230=DIRECTION('center_axis',(1.4081690688991E-16,0.,1.));
#117231=DIRECTION('ref_axis',(-1.,0.,1.4081690688991E-16));
#117232=DIRECTION('',(-1.,0.,1.40816906889911E-16));
#117233=DIRECTION('center_axis',(-1.4081690688991E-16,0.,-1.));
#117234=DIRECTION('ref_axis',(-1.,0.,1.4081690688991E-16));
#117235=DIRECTION('center_axis',(-1.4081690688991E-16,0.,-1.));
#117236=DIRECTION('ref_axis',(1.,0.,-1.4081690688991E-16));
#117237=DIRECTION('',(0.497266395846506,-0.0522601510654393,-0.86602252174666));
#117238=DIRECTION('center_axis',(-1.4081690688991E-16,0.,-1.));
#117239=DIRECTION('ref_axis',(-1.,0.,1.4081690688991E-16));
#117240=DIRECTION('center_axis',(-1.4081690688991E-16,0.,-1.));
#117241=DIRECTION('ref_axis',(-1.,0.,1.4081690688991E-16));
#117242=DIRECTION('center_axis',(-1.4081690688991E-16,0.,-1.));
#117243=DIRECTION('ref_axis',(-1.,0.,1.4081690688991E-16));
#117244=DIRECTION('',(-0.500004991781248,4.62770265298126E-6,0.866022521746645));
#117245=DIRECTION('center_axis',(-1.4081690688991E-16,0.,-1.));
#117246=DIRECTION('ref_axis',(-1.,0.,1.40816906889911E-16));
#117247=DIRECTION('',(0.994521895368273,-0.104528463267654,-1.40045497140051E-16));
#117248=DIRECTION('center_axis',(1.4081690688991E-16,0.,1.));
#117249=DIRECTION('ref_axis',(-1.,8.88178419700125E-16,1.4081690688991E-16));
#117250=DIRECTION('',(-1.,0.,1.40816906889911E-16));
#117251=DIRECTION('center_axis',(-1.4081690688991E-16,0.,-1.));
#117252=DIRECTION('ref_axis',(-1.,0.,1.40816906889911E-16));
#117253=DIRECTION('center_axis',(1.4081690688991E-16,0.,1.));
#117254=DIRECTION('ref_axis',(1.,0.,-1.40816906889911E-16));
#117255=DIRECTION('center_axis',(-1.4081690688991E-16,0.,-1.));
#117256=DIRECTION('ref_axis',(-1.,0.,1.17174841180864E-16));
#117257=DIRECTION('center_axis',(-0.10346401040769,-0.994633197962197,7.86457223164439E-6));
#117258=DIRECTION('ref_axis',(6.43152272453738E-7,-7.97390974138951E-6,
-0.999999999968001));
#117259=DIRECTION('center_axis',(0.00107025596496794,0.999999427244995,
7.86457231481231E-6));
#117260=DIRECTION('ref_axis',(-0.848044334090874,0.000911792658906122,-0.529924500330484));
#117261=DIRECTION('center_axis',(-1.4081690688991E-16,0.,-1.));
#117262=DIRECTION('ref_axis',(-1.,0.,1.13676889660403E-16));
#117263=DIRECTION('center_axis',(-0.103509373457973,-0.994628478131847,
-9.77058577218967E-6));
#117264=DIRECTION('ref_axis',(0.86994307128939,-0.090538327344475,0.484769908304186));
#117265=DIRECTION('center_axis',(0.00102464802306578,0.999999475000345,
-9.77051630226669E-6));
#117266=DIRECTION('ref_axis',(0.874648786634608,-0.000891471298440391,0.484756336026185));
#117267=DIRECTION('center_axis',(-1.4081690688991E-16,0.,-1.));
#117268=DIRECTION('ref_axis',(-1.,0.,1.15974593313694E-16));
#117269=DIRECTION('center_axis',(0.107112188925724,0.994246940479911,1.81624797797238E-5));
#117270=DIRECTION('ref_axis',(0.8602680136723,-0.0926692157703517,-0.501349539843035));
#117271=DIRECTION('center_axis',(0.0025982945487801,-0.999996624262643,
1.81316452304032E-5));
#117272=DIRECTION('ref_axis',(0.86697857380863,0.0022436375454785,-0.498340364256518));
#117273=DIRECTION('center_axis',(-1.4081690688991E-16,0.,-1.));
#117274=DIRECTION('ref_axis',(-1.,0.,1.16261524579732E-16));
#117275=DIRECTION('center_axis',(0.107125623152071,0.994245493086215,1.84940574365093E-5));
#117276=DIRECTION('ref_axis',(0.861991996922946,-0.0928851544029273,0.498339387699122));
#117277=DIRECTION('center_axis',(0.00261180600209789,-0.999996589057286,
1.85257109031372E-5));
#117278=DIRECTION('ref_axis',(0.865242466402697,0.0022691410444305,0.501348506861542));
#117279=DIRECTION('center_axis',(0.,0.,-1.));
#117280=DIRECTION('ref_axis',(-1.,0.,0.));
#117281=DIRECTION('',(1.,0.,0.));
#117282=DIRECTION('center_axis',(0.,0.,1.));
#117283=DIRECTION('ref_axis',(-1.,2.87680990140871E-12,0.));
#117284=DIRECTION('',(-1.,0.,0.));
#117285=DIRECTION('center_axis',(0.,0.,-1.));
#117286=DIRECTION('ref_axis',(-1.,0.,0.));
#117287=DIRECTION('center_axis',(0.,1.,0.));
#117288=DIRECTION('ref_axis',(0.,0.,1.));
#117289=DIRECTION('center_axis',(0.,1.,0.));
#117290=DIRECTION('ref_axis',(0.874651456243763,0.,-0.484752338922326));
#117291=DIRECTION('',(-0.529924709392054,0.,0.848044693619238));
#117292=DIRECTION('',(1.,0.,0.));
#117293=DIRECTION('',(-0.529924185123399,0.,-0.848045021223108));
#117294=DIRECTION('center_axis',(0.,1.,0.));
#117295=DIRECTION('ref_axis',(0.87464958095347,0.,0.484755722542725));
#117296=DIRECTION('',(-1.,0.,1.40816906889911E-16));
#117297=DIRECTION('',(-0.500005012714982,0.,0.866022509672752));
#117298=DIRECTION('center_axis',(9.46835263434497E-7,-0.999999999998207,
1.6399888684466E-6));
#117299=DIRECTION('ref_axis',(0.866072335964589,1.6672152936214E-10,-0.499918702267519));
#117300=DIRECTION('',(-1.,0.,1.40816906889911E-16));
#117301=DIRECTION('center_axis',(-9.46924650952009E-7,-0.999999999998207,
1.64014404584511E-6));
#117302=DIRECTION('ref_axis',(0.866043284546592,-5.6510002087391E-11,0.499969028332507));
#117303=DIRECTION('',(-0.500005169296824,0.,-0.866022419268955));
#117304=DIRECTION('',(-1.,0.,1.40816906889911E-16));
#117305=DIRECTION('center_axis',(0.,1.,0.));
#117306=DIRECTION('ref_axis',(0.,0.,1.));
#117307=DIRECTION('center_axis',(0.,-1.,0.));
#117308=DIRECTION('ref_axis',(0.874649580936389,0.,0.484755722573544));
#117309=DIRECTION('',(0.529924185123402,0.,0.848045021223106));
#117310=DIRECTION('',(-1.,0.,0.));
#117311=DIRECTION('',(0.529924709392048,0.,-0.848044693619242));
#117312=DIRECTION('center_axis',(0.,-1.,0.));
#117313=DIRECTION('ref_axis',(0.874651456263025,0.,-0.48475233888757));
#117314=DIRECTION('',(1.,0.,-1.40816906889911E-16));
#117315=DIRECTION('',(0.500005169296809,0.,0.866022419268964));
#117316=DIRECTION('center_axis',(-9.47055353975915E-7,0.999999999998206,
1.64037043322054E-6));
#117317=DIRECTION('ref_axis',(0.866072438648806,1.66973549937258E-10,0.499918524374633));
#117318=DIRECTION('',(1.,0.,-1.40816906889911E-16));
#117319=DIRECTION('center_axis',(9.46713288386241E-7,0.999999999998207,
1.63977759862047E-6));
#117320=DIRECTION('ref_axis',(0.866043178342335,-5.6270925409859E-11,-0.499969212298824));
#117321=DIRECTION('',(0.500005012714974,0.,-0.866022509672756));
#117322=DIRECTION('',(1.,0.,-1.40816906889911E-16));
#117323=DIRECTION('center_axis',(1.,0.,0.));
#117324=DIRECTION('ref_axis',(0.,0.,-1.));
#117325=DIRECTION('center_axis',(-1.,0.,0.));
#117326=DIRECTION('ref_axis',(0.,0.,1.));
#117327=DIRECTION('center_axis',(-0.50000501436341,0.,0.866022508721018));
#117328=DIRECTION('ref_axis',(0.,1.,0.));
#117329=DIRECTION('center_axis',(-0.866018223014682,-3.00422159123528E-5,
0.500012436349295));
#117330=DIRECTION('ref_axis',(0.500012217440787,-0.000989701289107013,0.866017784402437));
#117331=DIRECTION('center_axis',(0.500005023014372,-1.99980824065794E-14,
-0.866022503726316));
#117332=DIRECTION('ref_axis',(-0.866022503726316,2.47318747560494E-28,-0.500005023014372));
#117333=DIRECTION('center_axis',(1.,0.,0.));
#117334=DIRECTION('ref_axis',(0.,0.,-1.));
#117335=DIRECTION('center_axis',(-1.,0.,1.4081690688991E-16));
#117336=DIRECTION('ref_axis',(1.40816906889911E-16,0.,1.));
#117337=DIRECTION('center_axis',(-1.,0.,0.));
#117338=DIRECTION('ref_axis',(0.,0.,1.));
#117339=DIRECTION('center_axis',(-1.,0.,1.4081690688991E-16));
#117340=DIRECTION('ref_axis',(1.40816906889911E-16,0.,1.));
#117341=DIRECTION('center_axis',(1.,0.,0.));
#117342=DIRECTION('ref_axis',(0.,0.,-1.));
#117343=DIRECTION('center_axis',(-0.529924213265765,0.,-0.848045003637578));
#117344=DIRECTION('ref_axis',(-0.848045003637578,0.,0.529924213265765));
#117345=DIRECTION('center_axis',(0.500005158533463,0.,0.866022425483271));
#117346=DIRECTION('ref_axis',(0.866022425483271,0.,-0.500005158533463));
#117347=DIRECTION('center_axis',(0.529924185004324,-2.16262675490169E-8,
0.848045021297515));
#117348=DIRECTION('ref_axis',(0.848037146343382,-0.004309503024554,-0.529919264233199));
#117349=DIRECTION('center_axis',(-0.529924157141051,0.,-0.848045038708645));
#117350=DIRECTION('ref_axis',(-0.848045038708645,0.,0.529924157141051));
#117351=DIRECTION('center_axis',(0.500005172385364,-1.05122400740158E-8,
0.866022417485762));
#117352=DIRECTION('ref_axis',(0.866013458679462,-0.00454855867535886,-0.500000000000012));
#117353=DIRECTION('center_axis',(0.866037336481604,3.44576745566438E-5,
0.499979330205277));
#117354=DIRECTION('ref_axis',(0.499979069431793,0.000963977570940208,-0.866036951219381));
#117355=DIRECTION('center_axis',(-0.00024249581833115,-0.999999970597889,
-1.33391011393658E-17));
#117356=DIRECTION('ref_axis',(0.999999970597889,-0.00024249581833115,2.11314776580936E-36));
#117357=DIRECTION('center_axis',(-1.,0.,1.4081690688991E-16));
#117358=DIRECTION('ref_axis',(1.40816906889911E-16,0.,1.));
#117359=DIRECTION('center_axis',(1.,0.,0.));
#117360=DIRECTION('ref_axis',(0.,0.,-1.));
#117361=DIRECTION('center_axis',(0.,0.,-1.));
#117362=DIRECTION('ref_axis',(1.,-1.22464679914735E-16,0.));
#117363=DIRECTION('center_axis',(0.000242495818331158,-0.999999970597889,
0.));
#117364=DIRECTION('ref_axis',(0.999999970597889,0.000242495818331158,0.));
#117365=DIRECTION('center_axis',(0.529924676825566,-1.73811117043118E-14,
-0.848044713969328));
#117366=DIRECTION('ref_axis',(-0.848044713969328,2.32169098057144E-28,-0.529924676825566));
#117367=DIRECTION('center_axis',(0.529924157141051,0.,0.848045038708645));
#117368=DIRECTION('ref_axis',(0.848045038708645,0.,-0.529924157141051));
#117369=DIRECTION('center_axis',(0.529924709439987,2.52123003281154E-8,
-0.848044693589285));
#117370=DIRECTION('ref_axis',(-0.848035979777038,0.00453325469494587,-0.529919264233213));
#117371=DIRECTION('center_axis',(0.529924742154432,2.89534768729527E-14,
-0.848044673146739));
#117372=DIRECTION('ref_axis',(-0.848044673146739,-6.50756462101157E-28,
-0.529924742154432));
#117373=DIRECTION('center_axis',(-0.529924185162637,2.16871498834536E-8,
-0.848045021198589));
#117374=DIRECTION('ref_axis',(0.84803714634339,0.00430950302080326,-0.529919264233217));
#117375=DIRECTION('center_axis',(0.52992421326579,0.,0.848045003637563));
#117376=DIRECTION('ref_axis',(0.848045003637563,0.,-0.52992421326579));
#117377=DIRECTION('center_axis',(-0.000258180127964207,-0.99999996667151,
2.74452783786513E-17));
#117378=DIRECTION('ref_axis',(0.99999996667151,-0.000258180127964207,3.13697794718818E-34));
#117379=DIRECTION('center_axis',(1.,0.,0.));
#117380=DIRECTION('ref_axis',(0.,0.,-1.));
#117381=DIRECTION('center_axis',(0.,0.,-1.));
#117382=DIRECTION('ref_axis',(1.,-1.22464679914735E-16,0.));
#117383=DIRECTION('center_axis',(0.000258180127964191,-0.99999996667151,
-7.67076204667453E-19));
#117384=DIRECTION('ref_axis',(0.99999996667151,0.000258180127964191,6.2059328036136E-36));
#117385=DIRECTION('center_axis',(1.,0.,-1.4081690688991E-16));
#117386=DIRECTION('ref_axis',(-1.40816906889911E-16,0.,-1.));
#117387=DIRECTION('center_axis',(0.866018223015031,-3.00422149566322E-5,
-0.500012436348692));
#117388=DIRECTION('ref_axis',(0.500012217440177,0.000989701300755193,0.866017784402776));
#117389=DIRECTION('center_axis',(-0.529924742154432,2.89534768729527E-14,
0.848044673146739));
#117390=DIRECTION('ref_axis',(0.848044673146739,-6.50756462101157E-28,0.529924742154432));
#117391=DIRECTION('center_axis',(-0.500005009599423,-1.01154993436287E-8,
0.866022511471544));
#117392=DIRECTION('ref_axis',(-0.866013834616154,-0.00447641077897882,-0.499999999999963));
#117393=DIRECTION('center_axis',(0.50000502301429,0.,-0.866022503726363));
#117394=DIRECTION('ref_axis',(-0.866022503726363,0.,-0.50000502301429));
#117395=DIRECTION('center_axis',(-0.529924709245855,-2.52865664166506E-8,
0.848044693710594));
#117396=DIRECTION('ref_axis',(-0.848035979777064,-0.00453325468699187,-0.529919264233239));
#117397=DIRECTION('center_axis',(-0.529924676825566,0.,0.848044713969328));
#117398=DIRECTION('ref_axis',(0.848044713969328,0.,0.529924676825566));
#117399=DIRECTION('center_axis',(1.,0.,0.));
#117400=DIRECTION('ref_axis',(0.,0.,-1.));
#117401=DIRECTION('center_axis',(-1.,0.,0.));
#117402=DIRECTION('ref_axis',(0.,0.,1.));
#117403=DIRECTION('center_axis',(1.,0.,-1.4081690688991E-16));
#117404=DIRECTION('ref_axis',(-1.40816906889911E-16,0.,-1.));
#117405=DIRECTION('center_axis',(1.,0.,-5.46369598732844E-14));
#117406=DIRECTION('ref_axis',(-5.46369598732844E-14,0.,-1.));
#117407=DIRECTION('center_axis',(1.,0.,-1.4081690688991E-16));
#117408=DIRECTION('ref_axis',(-1.40816906889911E-16,0.,-1.));
#117409=DIRECTION('center_axis',(-0.866037336481684,3.44576748030691E-5,
-0.499979330205138));
#117410=DIRECTION('ref_axis',(0.499979069431657,-0.000963977564006246,-0.866036951219467));
#117411=DIRECTION('center_axis',(0.500005158533422,0.,0.866022425483294));
#117412=DIRECTION('ref_axis',(0.866022425483294,0.,-0.500005158533422));
#117413=DIRECTION('center_axis',(0.500005167510848,3.81405054986521E-20,
0.866022420300104));
#117414=DIRECTION('ref_axis',(-5.80463060321091E-12,-1.,3.35689480667619E-12));
#117415=DIRECTION('center_axis',(-7.71409749859041E-19,-1.47193748793066E-17,
-1.));
#117416=DIRECTION('ref_axis',(0.,1.,-1.47193748793066E-17));
#117417=DIRECTION('',(0.994521895368273,-0.104528463267654,7.71409749859047E-19));
#117418=DIRECTION('center_axis',(7.71409749859041E-19,1.47193748793066E-17,
1.));
#117419=DIRECTION('ref_axis',(-1.13546692937274E-35,1.,-1.47193748793066E-17));
#117420=DIRECTION('',(-0.994521895368273,0.104528463267654,-7.71409749859047E-19));
#117421=DIRECTION('center_axis',(-7.71409749859041E-19,-1.47193748793066E-17,
-1.));
#117422=DIRECTION('ref_axis',(-1.13546692937274E-35,1.,-1.47193748793066E-17));
#117423=DIRECTION('center_axis',(0.104528463267654,0.994521895368273,-1.47193748793066E-17));
#117424=DIRECTION('ref_axis',(7.71409749859047E-19,1.47193748793066E-17,
1.));
#117425=DIRECTION('center_axis',(0.104528463267658,0.994521895368273,9.44192068578644E-15));
#117426=DIRECTION('ref_axis',(0.869860024050839,-0.0914259726160459,-0.484752338921106));
#117427=DIRECTION('',(-0.527021726387054,0.0553922155203088,0.848044693619246));
#117428=DIRECTION('',(0.994521895368273,-0.104528463267654,7.71409749859047E-19));
#117429=DIRECTION('',(-0.527021204990396,0.0553921607193119,-0.848045021223117));
#117430=DIRECTION('center_axis',(0.104528463267649,0.994521895368274,9.30408455334034E-16));
#117431=DIRECTION('ref_axis',(0.869858159032171,-0.0914257765946819,0.484755722544067));
#117432=DIRECTION('',(-0.994521895368273,0.104528463267654,1.40045497140051E-16));
#117433=DIRECTION('',(-0.497265932938937,0.0522647556052235,0.866022509672754));
#117434=DIRECTION('center_axis',(-0.104527521619077,-0.994521994337724,
1.63998885004745E-6));
#117435=DIRECTION('ref_axis',(0.861327901104895,-0.090529210190981,-0.499918702271112));
#117436=DIRECTION('',(-0.994521895368273,0.104528463267654,1.40045497140051E-16));
#117437=DIRECTION('center_axis',(-0.10452940500478,-0.99452179638591,1.64014407352427E-6));
#117438=DIRECTION('ref_axis',(0.861299008811912,-0.0905261737130823,0.499969028333243));
#117439=DIRECTION('',(-0.497266088663009,0.0522647719724877,-0.866022419268957));
#117440=DIRECTION('',(-0.994521895368273,0.104528463267654,1.40045497140051E-16));
#117441=DIRECTION('center_axis',(0.104528463267654,0.994521895368273,-1.47193748793066E-17));
#117442=DIRECTION('ref_axis',(7.71409749859047E-19,1.47193748793066E-17,
1.));
#117443=DIRECTION('center_axis',(-0.10452846326766,-0.994521895368273,1.53689692974248E-14));
#117444=DIRECTION('ref_axis',(0.869858159016364,-0.0914257765930224,0.484755722572745));
#117445=DIRECTION('',(0.527021204990418,-0.0553921607193131,0.848045021223103));
#117446=DIRECTION('',(-0.994521895368273,0.104528463267654,-7.71409749859047E-19));
#117447=DIRECTION('',(0.527021726387064,-0.0553922155203084,-0.84804469361924));
#117448=DIRECTION('center_axis',(-0.104528463267655,-0.994521895368273,
-5.16893468263946E-15));
#117449=DIRECTION('ref_axis',(0.86986002406852,-0.0914259726179035,-0.484752338889029));
#117450=DIRECTION('',(0.994521895368273,-0.104528463267654,-1.40045497140051E-16));
#117451=DIRECTION('',(0.497266088663021,-0.0522647719724764,0.866022419268951));
#117452=DIRECTION('center_axis',(0.104527521400183,0.99452199436073,1.64037041736128E-6));
#117453=DIRECTION('ref_axis',(0.861328003227763,-0.0905292209242674,0.499918524376243));
#117454=DIRECTION('',(0.994521895368273,-0.104528463267654,-1.40045497140051E-16));
#117455=DIRECTION('center_axis',(0.104529404794558,0.994521796408006,1.6397775895808E-6));
#117456=DIRECTION('ref_axis',(0.861298903189669,-0.0905261626115,-0.499969212299227));
#117457=DIRECTION('',(0.497265932938941,-0.0522647556052202,-0.866022509672752));
#117458=DIRECTION('',(0.994521895368273,-0.104528463267654,-1.40045497140051E-16));
#117459=DIRECTION('center_axis',(-3.07718727278886E-18,-2.92774812072083E-17,
-1.));
#117460=DIRECTION('ref_axis',(0.,1.,-2.92774812072083E-17));
#117461=DIRECTION('',(0.978147600733805,-0.20791169081776,3.07718727278885E-18));
#117462=DIRECTION('center_axis',(3.07718727278886E-18,2.92774812072083E-17,
1.));
#117463=DIRECTION('ref_axis',(2.06146211212399E-12,1.,-2.92774812072147E-17));
#117464=DIRECTION('',(-0.978147600733805,0.20791169081776,-3.07718727278885E-18));
#117465=DIRECTION('center_axis',(-3.07718727278886E-18,-2.92774812072083E-17,
-1.));
#117466=DIRECTION('ref_axis',(-9.00922925501365E-35,1.,-2.92774812072083E-17));
#117467=DIRECTION('center_axis',(0.20791169081776,0.978147600733806,-2.92774812072083E-17));
#117468=DIRECTION('ref_axis',(3.07718727278885E-18,2.92774812072083E-17,
1.));
#117469=DIRECTION('center_axis',(0.20791169081775,0.978147600733808,-1.98487091788775E-14));
#117470=DIRECTION('ref_axis',(0.855538223403966,-0.181850263144028,-0.484752338920849));
#117471=DIRECTION('',(-0.518344583061404,0.110177542335813,0.848044693619234));
#117472=DIRECTION('',(0.978147600733806,-0.20791169081776,3.07718727278885E-18));
#117473=DIRECTION('',(-0.51834407024927,0.110177433334225,-0.848045021223109));
#117474=DIRECTION('center_axis',(0.207911690817753,0.978147600733807,2.06757434518666E-14));
#117475=DIRECTION('ref_axis',(0.855536389092489,-0.18184987324909,0.48475572254268));
#117476=DIRECTION('',(-0.978147600733806,0.20791169081776,1.37739719617122E-16));
#117477=DIRECTION('',(-0.489078703542049,0.103956887610924,0.866022509672744));
#117478=DIRECTION('center_axis',(-0.207910764672752,-0.978147797590171,
1.63998885404889E-6));
#117479=DIRECTION('ref_axis',(0.847146577520636,-0.180066563577866,-0.49991870226701));
#117480=DIRECTION('',(-0.978147600733806,0.20791169081776,1.37739719617122E-16));
#117481=DIRECTION('center_axis',(-0.207912617049446,-0.978147403855349,
1.64014403655927E-6));
#117482=DIRECTION('ref_axis',(0.847118160899391,-0.18006052366677,0.499969028332038));
#117483=DIRECTION('',(-0.489078856702209,0.10395692016612,-0.866022419268944));
#117484=DIRECTION('',(-0.978147600733806,0.20791169081776,1.37739719617122E-16));
#117485=DIRECTION('center_axis',(0.20791169081776,0.978147600733806,-2.92774812072083E-17));
#117486=DIRECTION('ref_axis',(3.07718727278885E-18,2.92774812072083E-17,
1.));
#117487=DIRECTION('center_axis',(-0.207911690817745,-0.978147600733809,
-2.96352322775435E-14));
#117488=DIRECTION('ref_axis',(0.855536389075761,-0.181849873245532,0.484755722573536));
#117489=DIRECTION('',(0.51834407024926,-0.110177433334229,0.848045021223114));
#117490=DIRECTION('',(-0.978147600733806,0.20791169081776,-3.07718727278885E-18));
#117491=DIRECTION('',(0.518344583061397,-0.110177542335811,-0.848044693619238));
#117492=DIRECTION('center_axis',(-0.207911690817741,-0.978147600733809,
3.58379471329602E-14));
#117493=DIRECTION('ref_axis',(0.855538223421254,-0.181850263147702,-0.48475233888896));
#117494=DIRECTION('',(0.978147600733806,-0.20791169081776,-1.37739719617122E-16));
#117495=DIRECTION('',(0.489078856702182,-0.103956920166122,0.866022419268959));
#117496=DIRECTION('center_axis',(0.207910764457463,0.978147797635931,1.64037042063162E-6));
#117497=DIRECTION('ref_axis',(0.847146677961002,-0.180066584926861,0.499918524374138));
#117498=DIRECTION('',(0.978147600733806,-0.20791169081776,-1.37739719617122E-16));
#117499=DIRECTION('center_axis',(0.207912616842747,0.978147403899286,1.63977763102226E-6));
#117500=DIRECTION('ref_axis',(0.847118057016918,-0.180060501585644,-0.499969212296724));
#117501=DIRECTION('',(0.489078703542038,-0.103956887610914,-0.866022509672751));
#117502=DIRECTION('',(0.978147600733806,-0.20791169081776,-1.37739719617122E-16));
#117503=DIRECTION('center_axis',(-6.89206998773325E-18,-4.35148173242971E-17,
-1.));
#117504=DIRECTION('ref_axis',(0.,1.,-4.35148173242971E-17));
#117505=DIRECTION('',(0.951056516295153,-0.309016994374948,6.89206998773323E-18));
#117506=DIRECTION('center_axis',(6.89206998773325E-18,4.35148173242971E-17,
1.));
#117507=DIRECTION('ref_axis',(-6.04138961080025E-12,1.,-4.35148173242554E-17));
#117508=DIRECTION('',(-0.951056516295153,0.309016994374948,-6.89206998773323E-18));
#117509=DIRECTION('center_axis',(-6.89206998773325E-18,-4.35148173242971E-17,
-1.));
#117510=DIRECTION('ref_axis',(-2.99907166502483E-34,1.,-4.3514817324297E-17));
#117511=DIRECTION('center_axis',(0.309016994374948,0.951056516295153,-4.35148173242971E-17));
#117512=DIRECTION('ref_axis',(6.89206998773323E-18,4.35148173242971E-17,
1.));
#117513=DIRECTION('center_axis',(0.309016994374967,0.951056516295147,1.64027527242141E-14));
#117514=DIRECTION('ref_axis',(0.831842966947326,-0.270282164134015,-0.484752338922984));
#117515=DIRECTION('',(-0.503988348013121,0.163755740941345,0.848044693619243));
#117516=DIRECTION('',(0.951056516295153,-0.309016994374948,6.89206998773323E-18));
#117517=DIRECTION('',(-0.503987849404001,0.163755578933424,-0.848045021223113));
#117518=DIRECTION('center_axis',(0.309016994374924,0.951056516295161,2.70163047771038E-14));
#117519=DIRECTION('ref_axis',(0.831841183440083,-0.270281584637364,0.484755722543754));
#117520=DIRECTION('',(-0.951056516295153,0.309016994374948,1.33924836902177E-16));
#117521=DIRECTION('',(-0.475533025522855,0.154510046201616,0.86602250967273));
#117522=DIRECTION('center_axis',(-0.309016093880578,-0.951056808881625,
1.63998878674474E-6));
#117523=DIRECTION('ref_axis',(0.823683738752414,-0.267631070012105,-0.4999187022697));
#117524=DIRECTION('',(-0.951056516295153,0.309016994374948,1.33924836902177E-16));
#117525=DIRECTION('center_axis',(-0.309017894953236,-0.951056223677644,
1.64014402270259E-6));
#117526=DIRECTION('ref_axis',(0.823656109144367,-0.267622092842979,0.499969028332263));
#117527=DIRECTION('',(-0.475533174441006,0.154510094588038,-0.866022419268956));
#117528=DIRECTION('',(-0.951056516295153,0.309016994374948,1.33924836902177E-16));
#117529=DIRECTION('center_axis',(0.309016994374948,0.951056516295153,-4.35148173242971E-17));
#117530=DIRECTION('ref_axis',(6.89206998773323E-18,4.35148173242971E-17,
1.));
#117531=DIRECTION('center_axis',(-0.309016994374939,-0.951056516295156,
-2.55000835876533E-14));
#117532=DIRECTION('ref_axis',(0.831841183424993,-0.270281584632475,0.484755722572375));
#117533=DIRECTION('',(0.50398784940402,-0.163755578933425,0.848045021223101));
#117534=DIRECTION('',(-0.951056516295153,0.309016994374948,-6.89206998773323E-18));
#117535=DIRECTION('',(0.503988348013121,-0.163755740941342,-0.848044693619244));
#117536=DIRECTION('center_axis',(-0.309016994374968,-0.951056516295147,
-3.11514463540405E-14));
#117537=DIRECTION('ref_axis',(0.831842966966041,-0.270282164140089,-0.484752338887482));
#117538=DIRECTION('',(0.951056516295153,-0.309016994374948,-1.33924836902177E-16));
#117539=DIRECTION('',(0.475533174441017,-0.154510094588048,0.866022419268948));
#117540=DIRECTION('center_axis',(0.309016093671225,0.951056808949647,1.64037048079197E-6));
#117541=DIRECTION('ref_axis',(0.823683836411307,-0.267631101743173,0.49991852437621));
#117542=DIRECTION('',(0.951056516295153,-0.309016994374948,-1.33924836902177E-16));
#117543=DIRECTION('center_axis',(0.309017894752217,0.95105622374296,1.63977757430429E-6));
#117544=DIRECTION('ref_axis',(0.823656008137434,-0.267622060023585,-0.499969212299957));
#117545=DIRECTION('',(0.475533025522778,-0.154510046201593,-0.866022509672777));
#117546=DIRECTION('',(0.951056516295153,-0.309016994374948,-1.33924836902177E-16));
#117547=DIRECTION('center_axis',(-1.21742612413517E-17,-5.72753959967198E-17,
-1.));
#117548=DIRECTION('ref_axis',(0.,1.,-5.72753959967198E-17));
#117549=DIRECTION('',(0.913545457642601,-0.406736643075801,1.21742612413517E-17));
#117550=DIRECTION('center_axis',(1.21742612413517E-17,5.72753959967198E-17,
1.));
#117551=DIRECTION('ref_axis',(6.46878029454758E-34,1.,-5.72753959967198E-17));
#117552=DIRECTION('',(-0.913545457642601,0.406736643075801,-1.21742612413517E-17));
#117553=DIRECTION('center_axis',(-1.21742612413517E-17,-5.72753959967198E-17,
-1.));
#117554=DIRECTION('ref_axis',(-6.97285633565939E-34,1.,-5.72753959967198E-17));
#117555=DIRECTION('center_axis',(0.406736643075801,0.913545457642601,-5.72753959967198E-17));
#117556=DIRECTION('ref_axis',(1.21742612413517E-17,5.72753959967198E-17,
1.));
#117557=DIRECTION('center_axis',(0.406736643075802,0.9135454576426,-1.92973561461323E-15));
#117558=DIRECTION('ref_axis',(0.799033864872045,-0.355752797173982,-0.484752338922186));
#117559=DIRECTION('',(-0.484110311157685,0.21553979738105,0.848044693619237));
#117560=DIRECTION('',(0.913545457642601,-0.406736643075801,1.21742612413517E-17));
#117561=DIRECTION('',(-0.48410983221443,0.215539584141768,-0.848045021223113));
#117562=DIRECTION('center_axis',(0.406736643075762,0.913545457642618,8.22894589384297E-14));
#117563=DIRECTION('ref_axis',(0.799032151707043,-0.355752034423781,0.48475572254668));
#117564=DIRECTION('',(-0.913545457642601,0.406736643075801,1.28642645648559E-16));
#117565=DIRECTION('',(-0.456777308164345,0.203370360392779,0.866022509672725));
#117566=DIRECTION('center_axis',(-0.406735778098035,-0.913545842753551,
1.63998882315082E-6));
#117567=DIRECTION('ref_axis',(0.791196448574938,-0.352263354437297,-0.499918702273668));
#117568=DIRECTION('',(-0.913545457642601,0.406736643075801,1.28642645648559E-16));
#117569=DIRECTION('center_axis',(-0.406737508133811,-0.913545072491997,
1.64014409189978E-6));
#117570=DIRECTION('ref_axis',(0.791169908697132,-0.352251538366759,0.49996902833118));
#117571=DIRECTION('',(-0.456777451208935,0.203370424080343,-0.866022419268953));
#117572=DIRECTION('',(-0.913545457642601,0.406736643075801,1.28642645648559E-16));
#117573=DIRECTION('center_axis',(0.406736643075801,0.913545457642601,-5.72753959967198E-17));
#117574=DIRECTION('ref_axis',(1.21742612413517E-17,5.72753959967198E-17,
1.));
#117575=DIRECTION('center_axis',(-0.406736643075822,-0.913545457642591,
5.01731374373309E-14));
#117576=DIRECTION('ref_axis',(0.799032151693804,-0.355752034417879,0.484755722572834));
#117577=DIRECTION('',(0.484109832214452,-0.215539584141766,0.848045021223101));
#117578=DIRECTION('',(-0.913545457642601,0.406736643075801,-1.21742612413517E-17));
#117579=DIRECTION('',(0.484110311157686,-0.215539797381044,-0.848044693619238));
#117580=DIRECTION('center_axis',(-0.406736643075838,-0.913545457642584,
-6.80920995526314E-14));
#117581=DIRECTION('ref_axis',(0.799033864889633,-0.355752797181813,-0.484752338887448));
#117582=DIRECTION('',(0.913545457642601,-0.406736643075801,-1.28642645648559E-16));
#117583=DIRECTION('',(0.456777451208942,-0.203370424080346,0.866022419268949));
#117584=DIRECTION('center_axis',(0.406735777896996,0.913545842843059,1.64037035504947E-6));
#117585=DIRECTION('ref_axis',(0.791196542384502,-0.352263396203737,0.499918524375541));
#117586=DIRECTION('',(0.913545457642601,-0.406736643075801,-1.28642645648559E-16));
#117587=DIRECTION('center_axis',(0.406737507940663,0.913545072577993,1.63977754573074E-6));
#117588=DIRECTION('ref_axis',(0.791169811676266,-0.352251495170018,-0.499969212294745));
#117589=DIRECTION('',(0.45677730816427,-0.203370360392744,-0.866022509672773));
#117590=DIRECTION('',(0.913545457642601,-0.406736643075801,-1.28642645648559E-16));
#117591=DIRECTION('center_axis',(-1.88658882409001E-17,-7.04084534449554E-17,
-1.));
#117592=DIRECTION('ref_axis',(0.,1.,-7.04084534449554E-17));
#117593=DIRECTION('',(0.866025403784438,-0.500000000000001,1.88658882409001E-17));
#117594=DIRECTION('center_axis',(1.88658882409001E-17,7.04084534449554E-17,
1.));
#117595=DIRECTION('ref_axis',(3.83604259468484E-12,1.,-7.04084534450278E-17));
#117596=DIRECTION('',(-0.866025403784438,0.500000000000001,-1.88658882409001E-17));
#117597=DIRECTION('center_axis',(-1.88658882409001E-17,-7.04084534449554E-17,
-1.));
#117598=DIRECTION('ref_axis',(8.89395021849247E-34,1.,-7.04084534449554E-17));
#117599=DIRECTION('center_axis',(0.500000000000001,0.866025403784438,-7.04084534449554E-17));
#117600=DIRECTION('ref_axis',(1.88658882409001E-17,7.04084534449554E-17,
1.));
#117601=DIRECTION('center_axis',(0.500000000000022,0.866025403784426,2.2605474342613E-14));
#117602=DIRECTION('ref_axis',(0.757470380563718,-0.437325728121644,-0.484752338923218));
#117603=DIRECTION('',(-0.458928260426596,0.264962354696016,0.848044693619246));
#117604=DIRECTION('',(0.866025403784438,-0.500000000000001,1.88658882409001E-17));
#117605=DIRECTION('',(-0.458927806396615,0.264962092561696,-0.848045021223118));
#117606=DIRECTION('center_axis',(0.500000000000048,0.866025403784411,-7.41569998473607E-14));
#117607=DIRECTION('ref_axis',(0.757468756513884,-0.437324790476036,0.484755722545285));
#117608=DIRECTION('',(-0.866025403784438,0.500000000000001,1.2195101864901E-16));
#117609=DIRECTION('',(-0.433017043030787,0.250002506357517,0.866022509672719));
#117610=DIRECTION('center_axis',(-0.499999180015722,-0.866025877200512,
1.63998882624894E-6));
#117611=DIRECTION('ref_axis',(0.750040644539098,-0.433036167835282,-0.499918702276589));
#117612=DIRECTION('',(-0.866025403784438,0.500000000000001,1.2195101864901E-16));
#117613=DIRECTION('center_axis',(-0.500000820059934,-0.866024930320544,
1.64014408122753E-6));
#117614=DIRECTION('ref_axis',(0.750015485167091,-0.433021642322871,0.499969028330332));
#117615=DIRECTION('',(-0.4330171786346,0.25000258464842,-0.866022419268947));
#117616=DIRECTION('',(-0.866025403784438,0.500000000000001,1.2195101864901E-16));
#117617=DIRECTION('center_axis',(0.500000000000001,0.866025403784438,-7.04084534449554E-17));
#117618=DIRECTION('ref_axis',(1.88658882409001E-17,7.04084534449554E-17,
1.));
#117619=DIRECTION('center_axis',(-0.499999999999992,-0.866025403784443,
-4.38325761128318E-14));
#117620=DIRECTION('ref_axis',(0.757468756499917,-0.437324790467973,0.484755722574385));
#117621=DIRECTION('',(0.458927806396625,-0.264962092561694,0.848045021223113));
#117622=DIRECTION('',(-0.866025403784438,0.500000000000001,-1.88658882409001E-17));
#117623=DIRECTION('',(0.458928260426603,-0.264962354696039,-0.848044693619235));
#117624=DIRECTION('center_axis',(-0.50000000000002,-0.866025403784427,-6.68515552287977E-14));
#117625=DIRECTION('ref_axis',(0.757470380581235,-0.437325728131731,-0.484752338886745));
#117626=DIRECTION('',(0.866025403784438,-0.500000000000001,-1.2195101864901E-16));
#117627=DIRECTION('',(0.433017178634607,-0.250002584648424,0.866022419268943));
#117628=DIRECTION('center_axis',(0.499999179825101,0.866025877310566,1.64037044197607E-6));
#117629=DIRECTION('ref_axis',(0.750040733470373,-0.433036219179497,0.499918524375674));
#117630=DIRECTION('',(0.866025403784438,-0.500000000000001,-1.2195101864901E-16));
#117631=DIRECTION('center_axis',(0.500000819876834,0.866024930426258,1.63977752249215E-6));
#117632=DIRECTION('ref_axis',(0.750015393194705,-0.433021589222314,-0.49996921229049));
#117633=DIRECTION('',(0.433017043030727,-0.250002506357485,-0.866022509672758));
#117634=DIRECTION('',(0.866025403784438,-0.500000000000001,-1.2195101864901E-16));
#117635=DIRECTION('center_axis',(-2.68936361206584E-17,-8.27701011433319E-17,
-1.));
#117636=DIRECTION('ref_axis',(0.,1.,-8.27701011433319E-17));
#117637=DIRECTION('',(0.809016994374947,-0.587785252292474,2.68936361206584E-17));
#117638=DIRECTION('center_axis',(2.68936361206584E-17,8.27701011433319E-17,
1.));
#117639=DIRECTION('ref_axis',(7.43345068374082E-34,1.,-8.27701011433319E-17));
#117640=DIRECTION('',(-0.809016994374947,0.587785252292474,-2.68936361206584E-17));
#117641=DIRECTION('center_axis',(-2.68936361206584E-17,-8.27701011433319E-17,
-1.));
#117642=DIRECTION('ref_axis',(9.35397677642635E-34,1.,-8.27701011433319E-17));
#117643=DIRECTION('center_axis',(0.587785252292474,0.809016994374947,-8.27701011433319E-17));
#117644=DIRECTION('ref_axis',(2.68936361206584E-17,8.27701011433319E-17,
1.));
#117645=DIRECTION('center_axis',(0.587785252292476,0.809016994374946,-3.44595645466632E-14));
#117646=DIRECTION('ref_axis',(0.707607892255973,-0.514107226876224,-0.48475233892236));
#117647=DIRECTION('',(-0.428718095637389,0.311481929006018,0.848044693619234));
#117648=DIRECTION('',(0.809016994374947,-0.587785252292474,2.68936361206584E-17));
#117649=DIRECTION('',(-0.42871767149514,0.311481620848648,-0.848045021223098));
#117650=DIRECTION('center_axis',(0.587785252292473,0.809016994374947,-1.4335182126627E-14));
#117651=DIRECTION('ref_axis',(0.707606375113141,-0.514106124607403,0.484755722545282));
#117652=DIRECTION('',(-0.809016994374947,0.587785252292474,1.13923270769252E-16));
#117653=DIRECTION('',(-0.404512552559106,0.293895572546189,0.866022509672736));
#117654=DIRECTION('center_axis',(-0.587784486285654,-0.809017550909262,
1.63998874706822E-6));
#117655=DIRECTION('ref_axis',(0.700667238248267,-0.509064546361347,-0.499918702274142));
#117656=DIRECTION('',(-0.809016994374947,0.587785252292474,1.13923270769252E-16));
#117657=DIRECTION('center_axis',(-0.587786018369519,-0.809016437785177,
1.64014399705464E-6));
#117658=DIRECTION('ref_axis',(0.70064373503004,-0.509047470549678,0.499969028330886));
#117659=DIRECTION('',(-0.404512679236429,0.29389566458273,-0.866022419268948));
#117660=DIRECTION('',(-0.809016994374947,0.587785252292474,1.13923270769252E-16));
#117661=DIRECTION('center_axis',(0.587785252292474,0.809016994374947,-8.27701011433319E-17));
#117662=DIRECTION('ref_axis',(2.68936361206584E-17,8.27701011433319E-17,
1.));
#117663=DIRECTION('center_axis',(-0.587785252292488,-0.809016994374937,
3.80433679469878E-14));
#117664=DIRECTION('ref_axis',(0.707606375100347,-0.514106124598112,0.484755722573811));
#117665=DIRECTION('',(0.428717671495134,-0.311481620848637,0.848045021223105));
#117666=DIRECTION('',(-0.809016994374947,0.587785252292474,-2.68936361206584E-17));
#117667=DIRECTION('',(0.428718095637378,-0.311481929006026,-0.848044693619237));
#117668=DIRECTION('center_axis',(-0.587785252292439,-0.809016994374972,
4.05244479118913E-14));
#117669=DIRECTION('ref_axis',(0.707607892271159,-0.514107226887212,-0.484752338888539));
#117670=DIRECTION('',(0.809016994374947,-0.587785252292474,-1.13923270769252E-16));
#117671=DIRECTION('',(0.404512679236463,-0.293895664582694,0.866022419268944));
#117672=DIRECTION('center_axis',(0.587784486107514,0.809017551038687,1.64037051564877E-6));
#117673=DIRECTION('ref_axis',(0.700667321323678,-0.509064606718872,0.499918524376984));
#117674=DIRECTION('',(0.809016994374947,-0.587785252292474,-1.13923270769252E-16));
#117675=DIRECTION('center_axis',(0.587786018198527,0.809016437909411,1.63977755536976E-6));
#117676=DIRECTION('ref_axis',(0.700643649105069,-0.509047408121237,-0.499969212305901));
#117677=DIRECTION('',(0.404512552559087,-0.293895572546175,-0.86602250967275));
#117678=DIRECTION('',(0.809016994374947,-0.587785252292474,-1.13923270769252E-16));
#117679=DIRECTION('center_axis',(-3.61695511949416E-17,-9.42249022928248E-17,
-1.));
#117680=DIRECTION('ref_axis',(0.,1.,-9.42249022928248E-17));
#117681=DIRECTION('',(0.743144825477393,-0.669130606358859,3.61695511949416E-17));
#117682=DIRECTION('center_axis',(3.61695511949416E-17,9.42249022928248E-17,
1.));
#117683=DIRECTION('ref_axis',(5.85418057251285E-34,1.,-9.42249022928248E-17));
#117684=DIRECTION('',(-0.743144825477393,0.669130606358859,-3.61695511949416E-17));
#117685=DIRECTION('center_axis',(-3.61695511949416E-17,-9.42249022928248E-17,
-1.));
#117686=DIRECTION('ref_axis',(8.43711753644579E-34,1.,-9.42249022928248E-17));
#117687=DIRECTION('center_axis',(0.669130606358859,0.743144825477393,-9.42249022928248E-17));
#117688=DIRECTION('ref_axis',(3.61695511949416E-17,9.42249022928248E-17,
1.));
#117689=DIRECTION('center_axis',(0.669130606358863,0.74314482547739,-2.5362239506344E-14));
#117690=DIRECTION('ref_axis',(0.649992703803064,-0.585256059268391,-0.484752338924131));
#117691=DIRECTION('',(-0.393810805677316,0.354588842120037,0.848044693619242));
#117692=DIRECTION('',(0.743144825477393,-0.669130606358859,3.61695511949416E-17));
#117693=DIRECTION('',(-0.393810416069769,0.354588491315839,-0.848045021223114));
#117694=DIRECTION('center_axis',(0.669130606358859,0.743144825477393,-4.13514869037259E-15));
#117695=DIRECTION('ref_axis',(0.649991310191181,-0.58525480445459,0.484755722543604));
#117696=DIRECTION('',(-0.743144825477393,0.669130606358859,1.04647355694969E-16));
#117697=DIRECTION('',(-0.371576137911905,0.334568657340474,0.866022509672737));
#117698=DIRECTION('center_axis',(-0.669129902721926,-0.743145459032521,
1.63998881471712E-6));
#117699=DIRECTION('ref_axis',(0.643617175073679,-0.579515507191499,-0.499918702265435));
#117700=DIRECTION('',(-0.743144825477393,0.669130606358859,1.04647355694969E-16));
#117701=DIRECTION('center_axis',(-0.669131310059734,-0.743144191859866,
1.64014392166056E-6));
#117702=DIRECTION('ref_axis',(0.643595585510885,-0.57949606816224,0.499969028336162));
#117703=DIRECTION('',(-0.371576254274916,0.334568762114208,-0.866022419268918));
#117704=DIRECTION('',(-0.743144825477393,0.669130606358859,1.04647355694969E-16));
#117705=DIRECTION('center_axis',(0.669130606358859,0.743144825477393,-9.42249022928248E-17));
#117706=DIRECTION('ref_axis',(3.61695511949416E-17,9.42249022928248E-17,
1.));
#117707=DIRECTION('center_axis',(-0.669130606358832,-0.743144825477418,
-7.1675910624755E-15));
#117708=DIRECTION('ref_axis',(0.649991310178681,-0.585254804443299,0.484755722573996));
#117709=DIRECTION('',(0.393810416069767,-0.35458849131585,0.848045021223111));
#117710=DIRECTION('',(-0.743144825477393,0.669130606358859,-3.61695511949416E-17));
#117711=DIRECTION('',(0.39381080567732,-0.354588842120049,-0.848044693619236));
#117712=DIRECTION('center_axis',(-0.669130606358823,-0.743144825477425,
4.43839191415929E-14));
#117713=DIRECTION('ref_axis',(0.649992703817898,-0.585256059281697,-0.484752338888176));
#117714=DIRECTION('',(0.743144825477393,-0.669130606358859,-1.04647355694969E-16));
#117715=DIRECTION('',(0.371576254274913,-0.334568762114135,0.866022419268947));
#117716=DIRECTION('center_axis',(0.669129902558282,0.743145459179866,1.64037065800196E-6));
#117717=DIRECTION('ref_axis',(0.6436172513831,-0.579515575900527,0.499918524372467));
#117718=DIRECTION('',(0.743144825477393,-0.669130606358859,-1.04647355694969E-16));
#117719=DIRECTION('center_axis',(0.669131309902781,0.743144192001188,1.63977770340336E-6));
#117720=DIRECTION('ref_axis',(0.643595506584037,-0.579495997095898,-0.499969212306785));
#117721=DIRECTION('',(0.3715761379119,-0.334568657340403,-0.866022509672767));
#117722=DIRECTION('',(0.743144825477393,-0.669130606358859,-1.04647355694969E-16));
#117723=DIRECTION('center_axis',(-4.6592004597086E-17,-1.04647355694969E-16,
-1.));
#117724=DIRECTION('ref_axis',(0.,1.,-1.04647355694969E-16));
#117725=DIRECTION('',(0.669130606358857,-0.743144825477395,4.6592004597086E-17));
#117726=DIRECTION('center_axis',(4.6592004597086E-17,1.04647355694969E-16,
1.));
#117727=DIRECTION('ref_axis',(3.5473846082823E-12,1.,-1.04647355695134E-16));
#117728=DIRECTION('',(-0.669130606358857,0.743144825477395,-4.6592004597086E-17));
#117729=DIRECTION('center_axis',(-4.6592004597086E-17,-1.04647355694969E-16,
-1.));
#117730=DIRECTION('ref_axis',(6.01228899222931E-34,1.,-1.04647355694969E-16));
#117731=DIRECTION('center_axis',(0.743144825477395,0.669130606358857,-1.04647355694969E-16));
#117732=DIRECTION('ref_axis',(4.6592004597086E-17,1.04647355694969E-16,
1.));
#117733=DIRECTION('center_axis',(0.74314482547737,0.669130606358885,-7.77407776172683E-14));
#117734=DIRECTION('ref_axis',(0.585256059269616,-0.64999270380446,-0.484752338920781));
#117735=DIRECTION('',(-0.354588842120056,0.393810805677302,0.848044693619241));
#117736=DIRECTION('',(0.669130606358857,-0.743144825477395,4.6592004597086E-17));
#117737=DIRECTION('',(-0.354588491315837,0.393810416069767,-0.848045021223116));
#117738=DIRECTION('center_axis',(0.743144825477371,0.669130606358884,3.94217508482209E-14));
#117739=DIRECTION('ref_axis',(0.585254804454593,-0.649991310191166,0.48475572254362));
#117740=DIRECTION('',(-0.669130606358857,0.743144825477395,9.42249022928245E-17));
#117741=DIRECTION('',(-0.33456865734047,0.371576137911935,0.866022509672725));
#117742=DIRECTION('center_axis',(-0.743144191919671,-0.669131309993315,
1.63998871109189E-6));
#117743=DIRECTION('ref_axis',(0.579515507438012,-0.643617174849089,-0.49991870226882));
#117744=DIRECTION('',(-0.669130606358857,0.743144825477395,9.42249022928245E-17));
#117745=DIRECTION('center_axis',(-0.743145459092338,-0.669129902655492,
1.64014408828484E-6));
#117746=DIRECTION('ref_axis',(0.579496068078453,-0.643595585586683,0.499969028335704));
#117747=DIRECTION('',(-0.334568762114167,0.371576254274909,-0.866022419268937));
#117748=DIRECTION('',(-0.669130606358857,0.743144825477395,9.42249022928245E-17));
#117749=DIRECTION('center_axis',(0.743144825477395,0.669130606358857,-1.04647355694969E-16));
#117750=DIRECTION('ref_axis',(4.6592004597086E-17,1.04647355694969E-16,
1.));
#117751=DIRECTION('center_axis',(-0.743144825477388,-0.669130606358865,
3.17028066224897E-14));
#117752=DIRECTION('ref_axis',(0.585254804443526,-0.649991310178857,0.484755722573486));
#117753=DIRECTION('',(0.354588491315847,-0.39381041606979,0.848045021223102));
#117754=DIRECTION('',(-0.669130606358857,0.743144825477395,-4.6592004597086E-17));
#117755=DIRECTION('',(0.354588842120031,-0.393810805677317,-0.848044693619244));
#117756=DIRECTION('center_axis',(-0.743144825477382,-0.669130606358872,
2.12270917633713E-14));
#117757=DIRECTION('ref_axis',(0.585256059282123,-0.649992703818332,-0.48475233888708));
#117758=DIRECTION('',(0.669130606358857,-0.743144825477395,-9.42249022928245E-17));
#117759=DIRECTION('',(0.334568762114171,-0.371576254274878,0.866022419268948));
#117760=DIRECTION('center_axis',(0.743144191772357,0.669131310156922,1.64037043440206E-6));
#117761=DIRECTION('ref_axis',(0.579515576147011,-0.643617251157822,0.49991852437677));
#117762=DIRECTION('',(0.669130606358857,-0.743144825477395,-9.42249022928245E-17));
#117763=DIRECTION('center_axis',(0.743145458950911,0.669129902812563,1.63977758704219E-6));
#117764=DIRECTION('ref_axis',(0.579495997015134,-0.643595506662556,-0.499969212299321));
#117765=DIRECTION('',(0.334568657340475,-0.371576137911903,-0.866022509672737));
#117766=DIRECTION('',(0.669130606358857,-0.743144825477395,-9.42249022928245E-17));
#117767=DIRECTION('center_axis',(-5.8046805746579E-17,-1.13923270769252E-16,
-1.));
#117768=DIRECTION('ref_axis',(0.,1.,-1.13923270769252E-16));
#117769=DIRECTION('',(0.587785252292471,-0.809016994374949,5.8046805746579E-17));
#117770=DIRECTION('center_axis',(5.8046805746579E-17,1.13923270769252E-16,
1.));
#117771=DIRECTION('ref_axis',(-2.03917556295434E-34,1.,-1.13923270769252E-16));
#117772=DIRECTION('',(-0.587785252292471,0.809016994374949,-5.8046805746579E-17));
#117773=DIRECTION('center_axis',(-5.8046805746579E-17,-1.13923270769252E-16,
-1.));
#117774=DIRECTION('ref_axis',(2.10605807273539E-34,1.,-1.13923270769252E-16));
#117775=DIRECTION('center_axis',(0.809016994374949,0.587785252292471,-1.13923270769252E-16));
#117776=DIRECTION('ref_axis',(5.8046805746579E-17,1.13923270769252E-16,
1.));
#117777=DIRECTION('center_axis',(0.809016994374928,0.5877852522925,-5.84434214711463E-14));
#117778=DIRECTION('ref_axis',(0.51410722687612,-0.707607892255862,-0.484752338922631));
#117779=DIRECTION('',(-0.311481929006011,0.428718095637375,0.848044693619244));
#117780=DIRECTION('',(0.587785252292471,-0.809016994374949,5.8046805746579E-17));
#117781=DIRECTION('',(-0.311481620848643,0.42871767149512,-0.84804502122311));
#117782=DIRECTION('center_axis',(0.809016994374939,0.587785252292485,3.91460742688633E-14));
#117783=DIRECTION('ref_axis',(0.514106124608326,-0.707606375114411,0.484755722542449));
#117784=DIRECTION('',(-0.587785252292471,0.809016994374949,8.27701011433315E-17));
#117785=DIRECTION('',(-0.293895572546222,0.404512552559057,0.866022509672748));
#117786=DIRECTION('center_axis',(-0.809016437837695,-0.587786018297235,
1.63998885723267E-6));
#117787=DIRECTION('ref_axis',(0.509064546631475,-0.70066723805277,-0.499918702273074));
#117788=DIRECTION('',(-0.587785252292471,0.809016994374949,8.27701011433315E-17));
#117789=DIRECTION('center_axis',(-0.809017550961851,-0.587784486213271,
1.64014409551461E-6));
#117790=DIRECTION('ref_axis',(0.509047470457721,-0.700643735095713,0.49996902833248));
#117791=DIRECTION('',(-0.293895664582671,0.404512679236479,-0.866022419268945));
#117792=DIRECTION('',(-0.587785252292471,0.809016994374949,8.27701011433315E-17));
#117793=DIRECTION('center_axis',(0.809016994374949,0.587785252292471,-1.13923270769252E-16));
#117794=DIRECTION('ref_axis',(5.8046805746579E-17,1.13923270769252E-16,
1.));
#117795=DIRECTION('center_axis',(-0.809016994374936,-0.587785252292489,
-1.90216839734942E-14));
#117796=DIRECTION('ref_axis',(0.514106124597937,-0.707606375100088,0.484755722574375));
#117797=DIRECTION('',(0.311481620848639,-0.428717671495141,0.8480450212231));
#117798=DIRECTION('',(-0.587785252292471,0.809016994374949,-5.8046805746579E-17));
#117799=DIRECTION('',(0.311481929006024,-0.428718095637357,-0.848044693619248));
#117800=DIRECTION('center_axis',(-0.809016994374946,-0.587785252292474,
-1.47486936277963E-14));
#117801=DIRECTION('ref_axis',(0.514107226887618,-0.707607892271675,-0.484752338887354));
#117802=DIRECTION('',(0.587785252292471,-0.809016994374949,-8.27701011433315E-17));
#117803=DIRECTION('',(0.29389566458269,-0.404512679236492,0.866022419268932));
#117804=DIRECTION('center_axis',(0.809016437708314,0.587786018475311,1.64037048466487E-6));
#117805=DIRECTION('ref_axis',(0.509064606988954,-0.700667321127302,0.499918524377196));
#117806=DIRECTION('',(0.587785252292471,-0.809016994374949,-8.27701011433315E-17));
#117807=DIRECTION('center_axis',(0.809017550837583,0.587784486384312,1.63977753368073E-6));
#117808=DIRECTION('ref_axis',(0.509047408033278,-0.700643649175448,-0.499969212296831));
#117809=DIRECTION('',(0.293895572546198,-0.404512552559071,-0.866022509672749));
#117810=DIRECTION('',(0.587785252292471,-0.809016994374949,-8.27701011433315E-17));
#117811=DIRECTION('center_axis',(-7.04084534449555E-17,-1.21951018649011E-16,
-1.));
#117812=DIRECTION('ref_axis',(0.,1.,-1.21951018649011E-16));
#117813=DIRECTION('',(0.499999999999998,-0.86602540378444,7.04084534449555E-17));
#117814=DIRECTION('center_axis',(7.04084534449556E-17,1.21951018649011E-16,
1.));
#117815=DIRECTION('ref_axis',(-8.12565151756264E-34,1.,-1.21951018649011E-16));
#117816=DIRECTION('',(-0.499999999999998,0.86602540378444,-7.04084534449555E-17));
#117817=DIRECTION('center_axis',(-7.04084534449556E-17,-1.21951018649011E-16,
-1.));
#117818=DIRECTION('ref_axis',(-3.09764893063087E-34,1.,-1.21951018649011E-16));
#117819=DIRECTION('center_axis',(0.86602540378444,0.499999999999998,-1.21951018649011E-16));
#117820=DIRECTION('ref_axis',(7.04084534449555E-17,1.21951018649011E-16,
1.));
#117821=DIRECTION('center_axis',(0.866025403784438,0.500000000000001,3.85947122922661E-15));
#117822=DIRECTION('ref_axis',(0.437325728121527,-0.757470380563533,-0.484752338923613));
#117823=DIRECTION('',(-0.264962354696013,0.458928260426604,0.848044693619243));
#117824=DIRECTION('',(0.499999999999998,-0.86602540378444,7.04084534449555E-17));
#117825=DIRECTION('',(-0.264962092561699,0.458927806396622,-0.848045021223113));
#117826=DIRECTION('center_axis',(0.866025403784433,0.50000000000001,2.81190110945387E-14));
#117827=DIRECTION('ref_axis',(0.437324790476745,-0.757468756515143,0.484755722542679));
#117828=DIRECTION('',(-0.499999999999998,0.86602540378444,7.04084534449549E-17));
#117829=DIRECTION('',(-0.250002506357482,0.433017043030748,0.866022509672748));
#117830=DIRECTION('center_axis',(-0.86602493036527,-0.500000819982468,1.63998884690466E-6));
#117831=DIRECTION('ref_axis',(0.433036168127082,-0.750040644377634,-0.499918702266075));
#117832=DIRECTION('',(-0.499999999999998,0.86602540378444,7.04084534449549E-17));
#117833=DIRECTION('center_axis',(-0.866025877245222,-0.499999179938281,
1.64014409947301E-6));
#117834=DIRECTION('ref_axis',(0.433021642224044,-0.750015485221962,0.499969028333613));
#117835=DIRECTION('',(-0.25000258464842,0.4330171786346,-0.866022419268947));
#117836=DIRECTION('',(-0.499999999999998,0.86602540378444,7.04084534449549E-17));
#117837=DIRECTION('center_axis',(0.86602540378444,0.499999999999998,-1.21951018649011E-16));
#117838=DIRECTION('ref_axis',(7.04084534449555E-17,1.21951018649011E-16,
1.));
#117839=DIRECTION('center_axis',(-0.866025403784437,-0.500000000000003,
4.96217842786824E-15));
#117840=DIRECTION('ref_axis',(0.437324790468618,-0.757468756501049,0.484755722572034));
#117841=DIRECTION('',(0.264962092561697,-0.458927806396632,0.848045021223108));
#117842=DIRECTION('',(-0.499999999999998,0.86602540378444,-7.04084534449555E-17));
#117843=DIRECTION('',(0.264962354696018,-0.4589282604266,-0.848044693619243));
#117844=DIRECTION('center_axis',(-0.866025403784433,-0.500000000000011,
3.28055054524852E-14));
#117845=DIRECTION('ref_axis',(0.437325728131414,-0.757470380580673,-0.484752338887911));
#117846=DIRECTION('',(0.499999999999998,-0.86602540378444,-7.04084534449549E-17));
#117847=DIRECTION('',(0.250002584648412,-0.433017178634587,0.866022419268956));
#117848=DIRECTION('center_axis',(0.866024930255237,0.500000820173048,1.64037033731929E-6));
#117849=DIRECTION('ref_axis',(0.433036219468869,-0.750040733303686,0.4999185243751));
#117850=DIRECTION('',(0.499999999999998,-0.86602540378444,-7.04084534449549E-17));
#117851=DIRECTION('center_axis',(0.866025877139543,0.499999180121325,1.63977763420594E-6));
#117852=DIRECTION('ref_axis',(0.433021589122406,-0.75001539324677,-0.499969212298916));
#117853=DIRECTION('',(0.250002506357476,-0.433017043030742,-0.866022509672753));
#117854=DIRECTION('',(0.499999999999998,-0.86602540378444,-7.04084534449549E-17));
#117855=DIRECTION('center_axis',(-8.35415108931911E-17,-1.28642645648559E-16,
-1.));
#117856=DIRECTION('ref_axis',(0.,1.,-1.28642645648559E-16));
#117857=DIRECTION('',(0.406736643075798,-0.913545457642602,8.35415108931911E-17));
#117858=DIRECTION('center_axis',(8.35415108931911E-17,1.28642645648559E-16,
1.));
#117859=DIRECTION('ref_axis',(-1.52315888917702E-33,1.,-1.28642645648559E-16));
#117860=DIRECTION('',(-0.406736643075798,0.913545457642602,-8.35415108931911E-17));
#117861=DIRECTION('center_axis',(-8.35415108931911E-17,-1.28642645648559E-16,
-1.));
#117862=DIRECTION('ref_axis',(-9.26572950507683E-34,1.,-1.28642645648559E-16));
#117863=DIRECTION('center_axis',(0.913545457642602,0.406736643075798,-1.28642645648559E-16));
#117864=DIRECTION('ref_axis',(8.35415108931911E-17,1.28642645648559E-16,
1.));
#117865=DIRECTION('center_axis',(0.913545457642591,0.406736643075822,-2.2329797826238E-14));
#117866=DIRECTION('ref_axis',(0.35575279717394,-0.799033864871932,-0.484752338922403));
#117867=DIRECTION('',(-0.215539797381028,0.48411031115768,0.848044693619245));
#117868=DIRECTION('',(0.406736643075798,-0.913545457642602,8.35415108931911E-17));
#117869=DIRECTION('',(-0.215539584141775,0.484109832214432,-0.84804502122311));
#117870=DIRECTION('center_axis',(0.913545457642603,0.406736643075797,-9.64868027753777E-16));
#117871=DIRECTION('ref_axis',(0.355752034424016,-0.799032151707585,0.484755722545614));
#117872=DIRECTION('',(-0.406736643075798,0.913545457642602,5.72753959967194E-17));
#117873=DIRECTION('',(-0.203370360392779,0.456777308164345,0.866022509672725));
#117874=DIRECTION('center_axis',(-0.913545072528371,-0.406737508052115,
1.63998885654379E-6));
#117875=DIRECTION('ref_axis',(0.352263354743201,-0.791196448442204,-0.499918702268187));
#117876=DIRECTION('',(-0.406736643075798,0.913545457642602,5.72753959967194E-17));
#117877=DIRECTION('center_axis',(-0.913545842789927,-0.406735778016334,
1.64014409086703E-6));
#117878=DIRECTION('ref_axis',(0.352251538262375,-0.791169908740555,0.499969028336008));
#117879=DIRECTION('',(-0.203370424080352,0.456777451208921,-0.866022419268959));
#117880=DIRECTION('',(-0.406736643075798,0.913545457642602,5.72753959967194E-17));
#117881=DIRECTION('center_axis',(0.913545457642602,0.406736643075798,-1.28642645648559E-16));
#117882=DIRECTION('ref_axis',(8.35415108931911E-17,1.28642645648559E-16,
1.));
#117883=DIRECTION('center_axis',(-0.913545457642604,-0.406736643075794,
2.75676579326004E-15));
#117884=DIRECTION('ref_axis',(0.355752034417364,-0.79903215169265,0.484755722575115));
#117885=DIRECTION('',(0.215539584141774,-0.484109832214442,0.848045021223105));
#117886=DIRECTION('',(-0.406736643075798,0.913545457642602,-8.35415108931911E-17));
#117887=DIRECTION('',(0.215539797381044,-0.484110311157686,-0.848044693619238));
#117888=DIRECTION('center_axis',(-0.913545457642585,-0.406736643075836,
6.54731726467594E-14));
#117889=DIRECTION('ref_axis',(0.355752797181805,-0.799033864889616,-0.484752338887483));
#117890=DIRECTION('',(0.406736643075798,-0.913545457642602,-5.72753959967194E-17));
#117891=DIRECTION('',(0.203370424080343,-0.456777451208935,0.866022419268953));
#117892=DIRECTION('center_axis',(0.91354507243885,0.40673750825318,1.64037042149229E-6));
#117893=DIRECTION('ref_axis',(0.352263396508779,-0.791196542248603,0.499918524375676));
#117894=DIRECTION('',(0.406736643075798,-0.913545457642602,-5.72753959967194E-17));
#117895=DIRECTION('center_axis',(0.913545842703946,0.406735778209453,1.63977757396033E-6));
#117896=DIRECTION('ref_axis',(0.352251495066729,-0.791169811720976,-0.499969212296767));
#117897=DIRECTION('',(0.203370360392771,-0.456777308164288,-0.866022509672757));
#117898=DIRECTION('',(0.406736643075798,-0.913545457642602,-5.72753959967194E-17));
#117899=DIRECTION('center_axis',(-9.73020895656139E-17,-1.33924836902177E-16,
-1.));
#117900=DIRECTION('ref_axis',(0.,1.,-1.33924836902177E-16));
#117901=DIRECTION('',(0.309016994374945,-0.951056516295154,9.73020895656138E-17));
#117902=DIRECTION('center_axis',(9.73020895656139E-17,1.33924836902177E-16,
1.));
#117903=DIRECTION('ref_axis',(-2.28801495776546E-33,1.,-1.33924836902177E-16));
#117904=DIRECTION('',(-0.309016994374945,0.951056516295154,-9.73020895656139E-17));
#117905=DIRECTION('center_axis',(-9.73020895656139E-17,-1.33924836902177E-16,
-1.));
#117906=DIRECTION('ref_axis',(-1.59316208980373E-33,1.,-1.33924836902177E-16));
#117907=DIRECTION('center_axis',(0.951056516295154,0.309016994374945,-1.33924836902177E-16));
#117908=DIRECTION('ref_axis',(9.73020895656139E-17,1.33924836902177E-16,
1.));
#117909=DIRECTION('center_axis',(0.95105651629516,0.309016994374929,2.49487247317848E-14));
#117910=DIRECTION('ref_axis',(0.270282164134087,-0.831842966947593,-0.484752338922485));
#117911=DIRECTION('',(-0.163755740941348,0.503988348013118,0.848044693619245));
#117912=DIRECTION('',(0.309016994374945,-0.951056516295154,9.73020895656139E-17));
#117913=DIRECTION('',(-0.163755578933429,0.503987849403997,-0.848045021223114));
#117914=DIRECTION('center_axis',(0.951056516295162,0.309016994374921,-3.08757768881175E-14));
#117915=DIRECTION('ref_axis',(0.270281584637474,-0.831841183440424,0.484755722543109));
#117916=DIRECTION('',(-0.309016994374945,0.951056516295154,4.35148173242966E-17));
#117917=DIRECTION('',(-0.15451004620159,0.475533025522823,0.866022509672753));
#117918=DIRECTION('center_axis',(-0.951056223705264,-0.309017894868233,
1.63998886704514E-6));
#117919=DIRECTION('ref_axis',(0.267631070329452,-0.823683738650044,-0.499918702268478));
#117920=DIRECTION('',(-0.309016994374945,0.951056516295154,4.35148173242966E-17));
#117921=DIRECTION('center_axis',(-0.951056808909262,-0.309016093795519,
1.64014407072764E-6));
#117922=DIRECTION('ref_axis',(0.267622092735341,-0.823656109178821,0.499969028333118));
#117923=DIRECTION('',(-0.154510094588055,0.475533174441005,-0.866022419268954));
#117924=DIRECTION('',(-0.309016994374945,0.951056516295154,4.35148173242966E-17));
#117925=DIRECTION('center_axis',(0.951056516295154,0.309016994374945,-1.33924836902177E-16));
#117926=DIRECTION('ref_axis',(9.73020895656139E-17,1.33924836902177E-16,
1.));
#117927=DIRECTION('center_axis',(-0.951056516295147,-0.309016994374967,
-3.33568660984481E-14));
#117928=DIRECTION('ref_axis',(0.270281584632006,-0.83184118342356,0.484755722575096));
#117929=DIRECTION('',(0.16375557893343,-0.503987849404013,0.848045021223104));
#117930=DIRECTION('',(-0.309016994374945,0.951056516295154,-9.73020895656139E-17));
#117931=DIRECTION('',(0.16375574094134,-0.503988348013128,-0.84804469361924));
#117932=DIRECTION('center_axis',(-0.951056516295154,-0.309016994374946,
-5.78920684455565E-15));
#117933=DIRECTION('ref_axis',(0.270282164139835,-0.831842966965265,-0.484752338888954));
#117934=DIRECTION('',(0.309016994374945,-0.951056516295154,-4.35148173242966E-17));
#117935=DIRECTION('',(0.154510094588053,-0.475533174441032,0.866022419268939));
#117936=DIRECTION('center_axis',(0.95105622363726,0.309017895077522,1.64037036907791E-6));
#117937=DIRECTION('ref_axis',(0.267631102060799,-0.823683836308256,0.499918524375959));
#117938=DIRECTION('',(0.309016994374945,-0.951056516295154,-4.35148173242966E-17));
#117939=DIRECTION('center_axis',(0.951056808843939,0.309016093996566,1.6397775629441E-6));
#117940=DIRECTION('ref_axis',(0.26762205991693,-0.823656008173377,-0.499969212297834));
#117941=DIRECTION('',(0.154510046201592,-0.475533025522835,-0.866022509672746));
#117942=DIRECTION('',(0.309016994374945,-0.951056516295154,-4.35148173242966E-17));
#117943=DIRECTION('center_axis',(-1.11539425682703E-16,-1.37739719617122E-16,
-1.));
#117944=DIRECTION('ref_axis',(0.,1.,-1.37739719617122E-16));
#117945=DIRECTION('',(0.207911690817756,-0.978147600733806,1.11539425682703E-16));
#117946=DIRECTION('center_axis',(1.11539425682703E-16,1.37739719617122E-16,
1.));
#117947=DIRECTION('ref_axis',(-3.0483093525691E-33,1.,-1.37739719617122E-16));
#117948=DIRECTION('',(-0.207911690817756,0.978147600733806,-1.11539425682703E-16));
#117949=DIRECTION('center_axis',(-1.11539425682703E-16,-1.37739719617122E-16,
-1.));
#117950=DIRECTION('ref_axis',(-2.25178493903976E-33,1.,-1.37739719617122E-16));
#117951=DIRECTION('center_axis',(0.978147600733806,0.207911690817756,-1.37739719617122E-16));
#117952=DIRECTION('ref_axis',(1.11539425682703E-16,1.37739719617122E-16,
1.));
#117953=DIRECTION('center_axis',(0.978147600733805,0.20791169081776,-2.48108864735987E-14));
#117954=DIRECTION('ref_axis',(0.181850263143634,-0.855538223402174,-0.484752338924158));
#117955=DIRECTION('',(-0.110177542335811,0.518344583061382,0.848044693619247));
#117956=DIRECTION('',(0.207911690817756,-0.978147600733806,1.11539425682703E-16));
#117957=DIRECTION('',(-0.110177433334228,0.518344070249267,-0.84804502122311));
#117958=DIRECTION('center_axis',(0.97814760073381,0.207911690817738,-2.55000835906321E-14));
#117959=DIRECTION('ref_axis',(0.181849873249065,-0.855536389092426,0.4847557225428));
#117960=DIRECTION('',(-0.207911690817756,0.978147600733806,2.92774812072079E-17));
#117961=DIRECTION('',(-0.103956887610938,0.489078703542067,0.866022509672732));
#117962=DIRECTION('center_axis',(-0.978147403873932,-0.207912616962023,
1.6399888759094E-6));
#117963=DIRECTION('ref_axis',(0.180066563904203,-0.84714657745219,-0.499918702265453));
#117964=DIRECTION('',(-0.207911690817756,0.978147600733806,2.92774812072079E-17));
#117965=DIRECTION('center_axis',(-0.978147797608757,-0.20791076458531,1.64014403328849E-6));
#117966=DIRECTION('ref_axis',(0.18006052355641,-0.847118160923773,0.499969028330471));
#117967=DIRECTION('',(-0.10395692016614,0.489078856702181,-0.866022419268957));
#117968=DIRECTION('',(-0.207911690817756,0.978147600733806,2.92774812072079E-17));
#117969=DIRECTION('center_axis',(0.978147600733806,0.207911690817756,-1.37739719617122E-16));
#117970=DIRECTION('ref_axis',(1.11539425682703E-16,1.37739719617122E-16,
1.));
#117971=DIRECTION('center_axis',(-0.978147600733803,-0.20791169081777,-9.51084198674744E-15));
#117972=DIRECTION('ref_axis',(0.181849873245419,-0.855536389075214,0.484755722574546));
#117973=DIRECTION('',(0.110177433334224,-0.518344070249276,0.848045021223105));
#117974=DIRECTION('',(-0.207911690817756,0.978147600733806,-1.11539425682703E-16));
#117975=DIRECTION('',(0.11017754233581,-0.518344583061379,-0.848044693619249));
#117976=DIRECTION('center_axis',(-0.978147600733808,-0.20791169081775,-3.85947122970341E-15));
#117977=DIRECTION('ref_axis',(0.18185026314786,-0.855538223422036,-0.484752338887519));
#117978=DIRECTION('',(0.207911690817756,-0.978147600733806,-2.92774812072079E-17));
#117979=DIRECTION('',(0.103956920166119,-0.489078856702202,0.866022419268949));
#117980=DIRECTION('center_axis',(0.978147403828174,0.207912617177293,1.64037041228311E-6));
#117981=DIRECTION('ref_axis',(0.180066585253765,-0.847146677892752,0.499918524372045));
#117982=DIRECTION('',(0.207911690817756,-0.978147600733806,-2.92774812072079E-17));
#117983=DIRECTION('center_axis',(0.978147797564809,0.207910764792073,1.63977756750503E-6));
#117984=DIRECTION('ref_axis',(0.180060501475011,-0.84711805703777,-0.499969212301239));
#117985=DIRECTION('',(0.103956887610919,-0.489078703542027,-0.866022509672757));
#117986=DIRECTION('',(0.207911690817756,-0.978147600733806,-2.92774812072079E-17));
#117987=DIRECTION('center_axis',(-1.26097532010604E-16,-1.40045497140051E-16,
-1.));
#117988=DIRECTION('ref_axis',(0.,1.,-1.40045497140051E-16));
#117989=DIRECTION('',(0.10452846326765,-0.994521895368274,1.26097532010604E-16));
#117990=DIRECTION('center_axis',(1.26097532010604E-16,1.40045497140051E-16,
1.));
#117991=DIRECTION('ref_axis',(-3.73692701101589E-33,1.,-1.40045497140052E-16));
#117992=DIRECTION('',(-0.10452846326765,0.994521895368274,-1.26097532010604E-16));
#117993=DIRECTION('center_axis',(-1.26097532010604E-16,-1.40045497140051E-16,
-1.));
#117994=DIRECTION('ref_axis',(-2.83644037037309E-33,1.,-1.40045497140051E-16));
#117995=DIRECTION('center_axis',(0.994521895368274,0.10452846326765,-1.40045497140051E-16));
#117996=DIRECTION('ref_axis',(1.26097532010604E-16,1.40045497140051E-16,
1.));
#117997=DIRECTION('center_axis',(0.994521895368275,0.10452846326764,2.23297978262382E-14));
#117998=DIRECTION('ref_axis',(0.091425972615977,-0.869860024050187,-0.48475233892229));
#117999=DIRECTION('',(-0.0553922155203048,0.527021726387063,0.848044693619241));
#118000=DIRECTION('',(0.10452846326765,-0.994521895368274,1.26097532010604E-16));
#118001=DIRECTION('',(-0.0553921607193106,0.5270212049904,-0.848045021223115));
#118002=DIRECTION('center_axis',(0.994521895368273,0.104528463267655,7.06421234605402E-15));
#118003=DIRECTION('ref_axis',(0.0914257765946829,-0.869858159032163,0.484755722544083));
#118004=DIRECTION('',(-0.10452846326765,0.994521895368274,1.47193748793061E-17));
#118005=DIRECTION('',(-0.0522647556052155,0.497265932938945,0.86602250967275));
#118006=DIRECTION('center_axis',(-0.994521796395255,-0.104529404915866,
1.63998885607056E-6));
#118007=DIRECTION('ref_axis',(0.0905292105227215,-0.86132790107118,-0.499918702269128));
#118008=DIRECTION('',(-0.10452846326765,0.994521895368274,1.47193748793061E-17));
#118009=DIRECTION('center_axis',(-0.994521994347068,-0.10452752153017,1.64014403010456E-6));
#118010=DIRECTION('ref_axis',(0.0905261736005623,-0.861299008822643,0.499969028335129));
#118011=DIRECTION('',(-0.0522647719724833,0.497266088663009,-0.866022419268957));
#118012=DIRECTION('',(-0.10452846326765,0.994521895368274,1.47193748793061E-17));
#118013=DIRECTION('center_axis',(0.994521895368274,0.10452846326765,-1.40045497140051E-16));
#118014=DIRECTION('ref_axis',(1.26097532010604E-16,1.40045497140051E-16,
1.));
#118015=DIRECTION('center_axis',(-0.994521895368273,-0.104528463267658,
-6.61623790382415E-15));
#118016=DIRECTION('ref_axis',(0.0914257765929248,-0.869858159015414,0.484755722574468));
#118017=DIRECTION('',(0.0553921607193095,-0.527021204990405,0.848045021223111));
#118018=DIRECTION('',(-0.10452846326765,0.994521895368274,-1.26097532010604E-16));
#118019=DIRECTION('',(0.0553922155203074,-0.52702172638707,-0.848044693619236));
#118020=DIRECTION('center_axis',(-0.994521895368274,-0.104528463267647,
-9.13178460599495E-15));
#118021=DIRECTION('ref_axis',(0.0914259726178967,-0.869860024068452,-0.484752338889152));
#118022=DIRECTION('',(0.10452846326765,-0.994521895368274,-1.47193748793061E-17));
#118023=DIRECTION('',(0.0522647719724736,-0.497266088663036,0.866022419268942));
#118024=DIRECTION('center_axis',(0.994521796372249,0.104529405134743,1.64037042463382E-6));
#118025=DIRECTION('ref_axis',(0.0905292212562927,-0.861328003191953,0.499918524377815));
#118026=DIRECTION('',(0.10452846326765,-0.994521895368274,-1.47193748793061E-17));
#118027=DIRECTION('center_axis',(0.994521994324975,0.104527521740383,1.63977756772086E-6));
#118028=DIRECTION('ref_axis',(0.0905261624998373,-0.861298903204019,-0.499969212294724));
#118029=DIRECTION('',(0.052264755605215,-0.497265932938933,-0.866022509672757));
#118030=DIRECTION('',(0.10452846326765,-0.994521895368274,-1.47193748793061E-17));
#118031=DIRECTION('center_axis',(-1.40816906889911E-16,-1.40816906889911E-16,
-1.));
#118032=DIRECTION('ref_axis',(-1.,-1.24216341050767E-48,1.40816906889911E-16));
#118033=DIRECTION('',(-3.49148133884313E-15,-1.,1.40816906889911E-16));
#118034=DIRECTION('center_axis',(1.40816906889911E-16,1.40816906889911E-16,
1.));
#118035=DIRECTION('ref_axis',(-1.,4.28176633132684E-33,1.40816906889911E-16));
#118036=DIRECTION('',(3.49148133884313E-15,1.,-1.40816906889911E-16));
#118037=DIRECTION('center_axis',(-1.40816906889911E-16,-1.40816906889911E-16,
-1.));
#118038=DIRECTION('ref_axis',(-1.,3.27616581394049E-33,1.40816906889911E-16));
#118039=DIRECTION('center_axis',(1.,-3.49148133884313E-15,-1.4081690688991E-16));
#118040=DIRECTION('ref_axis',(1.40816906889911E-16,1.40816906889911E-16,
1.));
#118041=DIRECTION('center_axis',(1.,-3.44043747061122E-15,-3.31073780200115E-16));
#118042=DIRECTION('ref_axis',(3.16967243309126E-15,0.87465145624295,0.484752338923792));
#118043=DIRECTION('',(1.96084725663077E-15,0.529924709392051,0.84804469361924));
#118044=DIRECTION('',(-3.49148133884313E-15,-1.,1.40816906889911E-16));
#118045=DIRECTION('',(1.75444295999834E-15,0.529924185123396,-0.84804502122311));
#118046=DIRECTION('center_axis',(1.,-3.58452992681196E-15,-2.19445148712539E-16));
#118047=DIRECTION('ref_axis',(3.02883030677949E-15,0.874649580953691,-0.484755722542326));
#118048=DIRECTION('',(3.49148133884313E-15,1.,-4.91659602599733E-31));
#118049=DIRECTION('',(1.92690513386533E-15,0.500005012715,0.866022509672741));
#118050=DIRECTION('center_axis',(-0.999999999998207,-9.468352603161E-7,
1.63998886905525E-6));
#118051=DIRECTION('ref_axis',(1.66718511939339E-10,-0.866072335961319,-0.499918702273184));
#118052=DIRECTION('',(3.49148133884313E-15,1.,-4.91659602599733E-31));
#118053=DIRECTION('center_axis',(-0.999999999998207,9.46924651316897E-7,
1.64014404046701E-6));
#118054=DIRECTION('ref_axis',(-5.65130098543586E-11,-0.866043284547351,
0.499969028331192));
#118055=DIRECTION('',(1.51399673284832E-15,0.50000516929684,-0.866022419268946));
#118056=DIRECTION('',(3.49148133884313E-15,1.,-4.91659602599733E-31));
#118057=DIRECTION('center_axis',(1.,-3.49148133884313E-15,-1.4081690688991E-16));
#118058=DIRECTION('ref_axis',(1.40816906889911E-16,1.40816906889911E-16,
1.));
#118059=DIRECTION('center_axis',(-1.,3.31723128487429E-15,-2.62780671920002E-16));
#118060=DIRECTION('ref_axis',(3.02879938767921E-15,0.87464958093635,-0.484755722573615));
#118061=DIRECTION('',(-1.70284169646898E-15,-0.529924185123411,0.8480450212231));
#118062=DIRECTION('',(3.49148133884313E-15,1.,-1.40816906889911E-16));
#118063=DIRECTION('',(-1.90924601303524E-15,-0.529924709392042,-0.848044693619246));
#118064=DIRECTION('center_axis',(-1.,3.24518402866523E-15,5.38039174125153E-16));
#118065=DIRECTION('ref_axis',(3.09922068458289E-15,0.874651456262602,0.484752338888334));
#118066=DIRECTION('',(-3.49148133884313E-15,-1.,4.91659602599733E-31));
#118067=DIRECTION('',(-1.65163279947087E-15,-0.500005169296866,0.866022419268931));
#118068=DIRECTION('center_axis',(0.999999999998206,9.47055346977043E-7,
1.64037042692596E-6));
#118069=DIRECTION('ref_axis',(1.66970631684952E-10,-0.866072438647882,0.499918524376234));
#118070=DIRECTION('',(-3.49148133884313E-15,-1.,4.91659602599733E-31));
#118071=DIRECTION('center_axis',(0.999999999998207,-9.46713286247913E-7,
1.63977758872445E-6));
#118072=DIRECTION('ref_axis',(-5.62740306604305E-11,-0.866043178344825,
-0.49996921229451));
#118073=DIRECTION('',(-1.92690513386536E-15,-0.500005012714974,-0.866022509672756));
#118074=DIRECTION('',(-3.49148133884313E-15,-1.,4.91659602599733E-31));
#118075=DIRECTION('center_axis',(-1.55536281769218E-16,-1.40045497140051E-16,
-1.));
#118076=DIRECTION('ref_axis',(-1.,3.43882990390064E-49,1.55536281769218E-16));
#118077=DIRECTION('',(-0.104528463267657,-0.994521895368273,1.55536281769218E-16));
#118078=DIRECTION('center_axis',(1.55536281769218E-16,1.40045497140051E-16,
1.));
#118079=DIRECTION('ref_axis',(-1.,6.31969253991851E-33,1.55536281769218E-16));
#118080=DIRECTION('',(0.104528463267657,0.994521895368273,-1.55536281769218E-16));
#118081=DIRECTION('center_axis',(-1.55536281769218E-16,-1.40045497140051E-16,
-1.));
#118082=DIRECTION('ref_axis',(-1.,5.31960080738412E-33,1.55536281769218E-16));
#118083=DIRECTION('center_axis',(0.994521895368273,-0.104528463267657,-1.40045497140051E-16));
#118084=DIRECTION('ref_axis',(1.55536281769218E-16,1.40045497140051E-16,
1.));
#118085=DIRECTION('center_axis',(0.994521895368273,-0.10452846326766,6.54731726386673E-15));
#118086=DIRECTION('ref_axis',(0.0914259726160302,0.869860024050657,0.484752338921436));
#118087=DIRECTION('',(0.055392215520309,0.52702172638707,0.848044693619236));
#118088=DIRECTION('',(-0.104528463267657,-0.994521895368273,1.55536281769218E-16));
#118089=DIRECTION('',(0.0553921607193155,0.527021204990399,-0.848045021223115));
#118090=DIRECTION('center_axis',(0.994521895368271,-0.104528463267675,-3.31156490954067E-14));
#118091=DIRECTION('ref_axis',(0.0914257765945625,0.869858159030975,-0.484755722546238));
#118092=DIRECTION('',(0.104528463267657,0.994521895368273,-1.47193748793071E-17));
#118093=DIRECTION('',(0.0522647556052243,0.497265932938944,0.866022509672749));
#118094=DIRECTION('center_axis',(-0.994521994337724,0.104527521619072,1.63998887332766E-6));
#118095=DIRECTION('ref_axis',(0.0905292101909773,0.861327901104786,0.499918702271301));
#118096=DIRECTION('',(0.104528463267657,0.994521895368273,-1.47193748793071E-17));
#118097=DIRECTION('center_axis',(-0.994521796385912,0.10452940500476,1.6401440452089E-6));
#118098=DIRECTION('ref_axis',(0.0905261737131933,0.861299008813,-0.499969028331347));
#118099=DIRECTION('',(0.0522647719724817,0.497266088662994,-0.866022419268966));
#118100=DIRECTION('',(0.104528463267657,0.994521895368273,-1.47193748793071E-17));
#118101=DIRECTION('center_axis',(0.994521895368273,-0.104528463267657,-1.40045497140051E-16));
#118102=DIRECTION('ref_axis',(1.55536281769218E-16,1.40045497140051E-16,
1.));
#118103=DIRECTION('center_axis',(-0.994521895368273,0.104528463267655,-3.51487638640649E-15));
#118104=DIRECTION('ref_axis',(0.0914257765928257,0.869858159014446,-0.484755722576225));
#118105=DIRECTION('',(-0.0553921607193145,-0.527021204990405,0.848045021223111));
#118106=DIRECTION('',(0.104528463267657,0.994521895368273,-1.55536281769218E-16));
#118107=DIRECTION('',(-0.0553922155203081,-0.527021726387063,-0.84804469361924));
#118108=DIRECTION('center_axis',(-0.994521895368272,0.104528463267671,-1.61615357743855E-14));
#118109=DIRECTION('ref_axis',(0.0914259726178233,0.869860024067671,0.484752338890568));
#118110=DIRECTION('',(-0.104528463267657,-0.994521895368273,1.47193748793071E-17));
#118111=DIRECTION('',(-0.0522647719724884,-0.497266088663051,0.866022419268933));
#118112=DIRECTION('center_axis',(0.99452199436073,-0.104527521400184,1.64037042497792E-6));
#118113=DIRECTION('ref_axis',(0.0905292209242248,0.861328003227316,-0.499918524377021));
#118114=DIRECTION('',(-0.104528463267657,-0.994521895368273,1.47193748793071E-17));
#118115=DIRECTION('center_axis',(0.994521796408007,-0.104529404794542,1.63977756733249E-6));
#118116=DIRECTION('ref_axis',(0.0905261626114006,0.861298903188755,0.49996921230082));
#118117=DIRECTION('',(-0.052264755605229,-0.49726593293894,-0.866022509672752));
#118118=DIRECTION('',(-0.104528463267657,-0.994521895368273,1.47193748793071E-17));
#118119=DIRECTION('center_axis',(-1.70094388097119E-16,-1.37739719617122E-16,
-1.));
#118120=DIRECTION('ref_axis',(-1.,6.23562738597969E-50,1.70094388097119E-16));
#118121=DIRECTION('',(-0.207911690817763,-0.978147600733805,1.70094388097119E-16));
#118122=DIRECTION('center_axis',(1.70094388097119E-16,1.37739719617122E-16,
1.));
#118123=DIRECTION('ref_axis',(-1.,-6.98701029200995E-33,1.70094388097119E-16));
#118124=DIRECTION('',(0.207911690817763,0.978147600733805,-1.70094388097119E-16));
#118125=DIRECTION('center_axis',(-1.70094388097119E-16,-1.37739719617122E-16,
-1.));
#118126=DIRECTION('ref_axis',(-1.,7.23724578308843E-33,1.70094388097119E-16));
#118127=DIRECTION('center_axis',(0.978147600733805,-0.207911690817763,-1.37739719617122E-16));
#118128=DIRECTION('ref_axis',(1.70094388097119E-16,1.37739719617122E-16,
1.));
#118129=DIRECTION('center_axis',(0.978147600733804,-0.207911690817767,2.10892535025602E-14));
#118130=DIRECTION('ref_axis',(0.181850263143708,0.855538223402485,0.484752338923582));
#118131=DIRECTION('',(0.110177542335813,0.518344583061401,0.848044693619235));
#118132=DIRECTION('',(-0.207911690817763,-0.978147600733805,1.70094388097119E-16));
#118133=DIRECTION('',(0.11017743333423,0.518344070249263,-0.848045021223112));
#118134=DIRECTION('center_axis',(0.9781476007338,-0.207911690817786,-3.70784999236818E-14));
#118135=DIRECTION('ref_axis',(0.181849873248753,0.855536389090898,-0.484755722545614));
#118136=DIRECTION('',(0.207911690817763,0.978147600733805,-2.92774812072088E-17));
#118137=DIRECTION('',(0.10395688761095,0.489078703542082,0.866022509672723));
#118138=DIRECTION('center_axis',(-0.978147797590169,0.207910764672762,1.63998886609772E-6));
#118139=DIRECTION('ref_axis',(0.18006656357774,0.847146577519975,0.499918702268176));
#118140=DIRECTION('',(0.207911690817763,0.978147600733805,-2.92774812072088E-17));
#118141=DIRECTION('center_axis',(-0.978147403855348,0.207912617049453,1.64014401168597E-6));
#118142=DIRECTION('ref_axis',(0.180060523666507,0.847118160898064,-0.499969028334382));
#118143=DIRECTION('',(0.10395692016612,0.489078856702209,-0.866022419268944));
#118144=DIRECTION('',(0.207911690817763,0.978147600733805,-2.92774812072088E-17));
#118145=DIRECTION('center_axis',(0.978147600733805,-0.207911690817763,-1.37739719617122E-16));
#118146=DIRECTION('ref_axis',(1.70094388097119E-16,1.37739719617122E-16,
1.));
#118147=DIRECTION('center_axis',(-0.978147600733803,0.207911690817772,1.15784163316921E-14));
#118148=DIRECTION('ref_axis',(0.181849873245457,0.855536389075389,-0.484755722574222));
#118149=DIRECTION('',(-0.110177433334229,-0.518344070249272,0.848045021223106));
#118150=DIRECTION('',(0.207911690817763,0.978147600733805,-1.70094388097119E-16));
#118151=DIRECTION('',(-0.110177542335815,-0.518344583061397,-0.848044693619238));
#118152=DIRECTION('center_axis',(-0.978147600733803,0.207911690817772,-2.01243856977405E-14));
#118153=DIRECTION('ref_axis',(0.181850263148122,0.855538223423227,0.48475233888532));
#118154=DIRECTION('',(-0.207911690817763,-0.978147600733805,2.92774812072088E-17));
#118155=DIRECTION('',(-0.103956920166122,-0.489078856702182,0.866022419268959));
#118156=DIRECTION('center_axis',(0.978147797635933,-0.207910764457452,1.6403704604808E-6));
#118157=DIRECTION('ref_axis',(0.180066584926772,0.847146677960533,-0.499918524374965));
#118158=DIRECTION('',(-0.207911690817763,-0.978147600733805,2.92774812072088E-17));
#118159=DIRECTION('center_axis',(0.978147403899289,-0.207912616842733,1.63977762473961E-6));
#118160=DIRECTION('ref_axis',(0.180060501584972,0.847118057013803,0.499969212302246));
#118161=DIRECTION('',(-0.103956887610927,-0.489078703542019,-0.866022509672761));
#118162=DIRECTION('',(-0.207911690817763,-0.978147600733805,2.92774812072088E-17));
#118163=DIRECTION('center_axis',(-1.84331724214208E-16,-1.33924836902177E-16,
-1.));
#118164=DIRECTION('ref_axis',(-1.,3.96466909511285E-49,1.84331724214208E-16));
#118165=DIRECTION('',(-0.309016994374951,-0.951056516295152,1.84331724214208E-16));
#118166=DIRECTION('center_axis',(1.84331724214208E-16,1.33924836902177E-16,
1.));
#118167=DIRECTION('ref_axis',(-1.,-4.8867629339927E-33,1.84331724214208E-16));
#118168=DIRECTION('',(0.309016994374951,0.951056516295152,-1.84331724214208E-16));
#118169=DIRECTION('center_axis',(-1.84331724214208E-16,-1.33924836902177E-16,
-1.));
#118170=DIRECTION('ref_axis',(-1.,-6.79952878369283E-33,1.84331724214208E-16));
#118171=DIRECTION('center_axis',(0.951056516295152,-0.309016994374951,-1.33924836902177E-16));
#118172=DIRECTION('ref_axis',(1.84331724214208E-16,1.33924836902177E-16,
1.));
#118173=DIRECTION('center_axis',(0.951056516295147,-0.309016994374967,1.64027527242136E-14));
#118174=DIRECTION('ref_axis',(0.270282164134392,0.831842966948485,0.484752338920785));
#118175=DIRECTION('',(0.163755740941359,0.503988348013124,0.848044693619239));
#118176=DIRECTION('',(-0.309016994374951,-0.951056516295152,1.84331724214208E-16));
#118177=DIRECTION('',(0.163755578933429,0.50398784940401,-0.848045021223106));
#118178=DIRECTION('center_axis',(0.951056516295152,-0.309016994374951,-1.48865352853428E-14));
#118179=DIRECTION('ref_axis',(0.270281584637258,0.831841183439741,-0.4847557225444));
#118180=DIRECTION('',(0.309016994374951,0.951056516295152,-4.35148173242975E-17));
#118181=DIRECTION('',(0.154510046201612,0.475533025522836,0.866022509672741));
#118182=DIRECTION('center_axis',(-0.951056808881645,0.309016093880519,1.63998890568801E-6));
#118183=DIRECTION('ref_axis',(0.267631070012908,0.823683738754867,0.499918702265228));
#118184=DIRECTION('',(0.309016994374951,0.951056516295152,-4.35148173242975E-17));
#118185=DIRECTION('center_axis',(-0.951056223677645,0.309017894953234,1.64014401443984E-6));
#118186=DIRECTION('ref_axis',(0.267622092842512,0.823656109142922,-0.499969028334893));
#118187=DIRECTION('',(0.154510094588035,0.475533174441033,-0.866022419268941));
#118188=DIRECTION('',(0.309016994374951,0.951056516295152,-4.35148173242975E-17));
#118189=DIRECTION('center_axis',(0.951056516295152,-0.309016994374951,-1.33924836902177E-16));
#118190=DIRECTION('ref_axis',(1.84331724214208E-16,1.33924836902177E-16,
1.));
#118191=DIRECTION('center_axis',(-0.951056516295152,0.309016994374953,-1.41973438352885E-14));
#118192=DIRECTION('ref_axis',(0.270281584632026,0.831841183423588,-0.484755722575036));
#118193=DIRECTION('',(-0.163755578933429,-0.50398784940401,0.848045021223106));
#118194=DIRECTION('',(0.309016994374951,0.951056516295152,-1.84331724214208E-16));
#118195=DIRECTION('',(-0.163755740941351,-0.50398834801313,-0.848044693619237));
#118196=DIRECTION('center_axis',(-0.951056516295161,0.309016994374925,4.4108242625183E-14));
#118197=DIRECTION('ref_axis',(0.270282164140163,0.831842966966275,0.484752338887038));
#118198=DIRECTION('',(-0.309016994374951,-0.951056516295152,4.35148173242975E-17));
#118199=DIRECTION('',(-0.15451009458806,-0.475533174441019,0.866022419268945));
#118200=DIRECTION('center_axis',(0.951056808949636,-0.30901609367126,1.64037036907829E-6));
#118201=DIRECTION('ref_axis',(0.267631101743422,0.823683836412152,-0.499918524374684));
#118202=DIRECTION('',(-0.309016994374951,-0.951056516295152,4.35148173242975E-17));
#118203=DIRECTION('center_axis',(0.951056223742969,-0.309017894752189,1.63977748978694E-6));
#118204=DIRECTION('ref_axis',(0.267622060023532,0.823656008137218,0.499969212300342));
#118205=DIRECTION('',(-0.154510046201597,-0.475533025522832,-0.866022509672746));
#118206=DIRECTION('',(-0.309016994374951,-0.951056516295152,4.35148173242975E-17));
#118207=DIRECTION('center_axis',(-1.98092302886631E-16,-1.28642645648559E-16,
-1.));
#118208=DIRECTION('ref_axis',(-1.,-1.14441315467514E-48,1.98092302886631E-16));
#118209=DIRECTION('',(-0.406736643075804,-0.913545457642599,1.98092302886631E-16));
#118210=DIRECTION('center_axis',(1.98092302886631E-16,1.28642645648559E-16,
1.));
#118211=DIRECTION('ref_axis',(-1.,-2.92382461743668E-33,1.98092302886631E-16));
#118212=DIRECTION('',(0.406736643075804,0.913545457642599,-1.98092302886631E-16));
#118213=DIRECTION('center_axis',(-1.98092302886631E-16,-1.28642645648559E-16,
-1.));
#118214=DIRECTION('ref_axis',(-1.,-4.76114818715937E-33,1.98092302886631E-16));
#118215=DIRECTION('center_axis',(0.913545457642599,-0.406736643075804,-1.28642645648559E-16));
#118216=DIRECTION('ref_axis',(1.98092302886631E-16,1.28642645648559E-16,
1.));
#118217=DIRECTION('center_axis',(0.913545457642599,-0.406736643075804,8.27029549119849E-16));
#118218=DIRECTION('ref_axis',(0.355752797173883,0.79903386487182,0.48475233892263));
#118219=DIRECTION('',(0.21553979738105,0.484110311157685,0.848044693619237));
#118220=DIRECTION('',(-0.406736643075804,-0.913545457642599,1.98092302886631E-16));
#118221=DIRECTION('',(0.215539584141768,0.48410983221443,-0.848045021223113));
#118222=DIRECTION('center_axis',(0.913545457642593,-0.406736643075818,-2.34325092454487E-14));
#118223=DIRECTION('ref_axis',(0.355752034424554,0.799032151708775,-0.484755722543257));
#118224=DIRECTION('',(0.406736643075804,0.913545457642599,-5.72753959967203E-17));
#118225=DIRECTION('',(0.203370360392782,0.456777308164353,0.866022509672721));
#118226=DIRECTION('center_axis',(-0.913545842753543,0.406735778098055,1.63998883055243E-6));
#118227=DIRECTION('ref_axis',(0.352263354438993,0.791196448578691,0.499918702266534));
#118228=DIRECTION('',(0.406736643075804,0.913545457642599,-5.72753959967203E-17));
#118229=DIRECTION('center_axis',(-0.913545072491979,0.406737508133851,1.64014412908005E-6));
#118230=DIRECTION('ref_axis',(0.352251538366349,0.791169908696165,-0.499969028332998));
#118231=DIRECTION('',(0.203370424080349,0.456777451208949,-0.866022419268945));
#118232=DIRECTION('',(0.406736643075804,0.913545457642599,-5.72753959967203E-17));
#118233=DIRECTION('center_axis',(0.913545457642599,-0.406736643075804,-1.28642645648559E-16));
#118234=DIRECTION('ref_axis',(1.98092302886631E-16,1.28642645648559E-16,
1.));
#118235=DIRECTION('center_axis',(-0.913545457642582,0.406736643075842,7.41569998386918E-14));
#118236=DIRECTION('ref_axis',(0.355752034417934,0.799032151693907,-0.484755722572623));
#118237=DIRECTION('',(-0.215539584141773,-0.484109832214439,0.848045021223107));
#118238=DIRECTION('',(0.406736643075804,0.913545457642599,-1.98092302886631E-16));
#118239=DIRECTION('',(-0.215539797381042,-0.48411031115768,-0.848044693619242));
#118240=DIRECTION('center_axis',(-0.913545457642587,0.406736643075831,-3.9559580104464E-14));
#118241=DIRECTION('ref_axis',(0.355752797181886,0.799033864889778,0.484752338887155));
#118242=DIRECTION('',(-0.406736643075804,-0.913545457642599,5.72753959967203E-17));
#118243=DIRECTION('',(-0.203370424080353,-0.456777451208954,0.866022419268941));
#118244=DIRECTION('center_axis',(0.913545842843099,-0.406735777896905,1.64037054559977E-6));
#118245=DIRECTION('ref_axis',(0.352263396203069,0.791196542382979,-0.499918524378422));
#118246=DIRECTION('',(-0.406736643075804,-0.913545457642599,5.72753959967203E-17));
#118247=DIRECTION('center_axis',(0.913545072577997,-0.406737507940653,1.63977751543501E-6));
#118248=DIRECTION('ref_axis',(0.352251495169236,0.791169811674494,0.4999692122981));
#118249=DIRECTION('',(-0.203370360392794,-0.4567773081643,-0.866022509672746));
#118250=DIRECTION('',(-0.406736643075804,-0.913545457642599,5.72753959967203E-17));
#118251=DIRECTION('center_axis',(-2.11225360334866E-16,-1.2195101864901E-16,
-1.));
#118252=DIRECTION('ref_axis',(-1.,-1.3208785554854E-48,2.11225360334866E-16));
#118253=DIRECTION('',(-0.500000000000004,-0.866025403784436,2.11225360334866E-16));
#118254=DIRECTION('center_axis',(2.11225360334866E-16,1.2195101864901E-16,
1.));
#118255=DIRECTION('ref_axis',(-1.,-1.17014578711787E-33,2.11225360334866E-16));
#118256=DIRECTION('',(0.500000000000004,0.866025403784436,-2.11225360334866E-16));
#118257=DIRECTION('center_axis',(-2.11225360334866E-16,-1.2195101864901E-16,
-1.));
#118258=DIRECTION('ref_axis',(-1.,-2.91189697534857E-33,2.11225360334866E-16));
#118259=DIRECTION('center_axis',(0.866025403784436,-0.500000000000004,-1.2195101864901E-16));
#118260=DIRECTION('ref_axis',(2.11225360334866E-16,1.2195101864901E-16,
1.));
#118261=DIRECTION('center_axis',(0.866025403784421,-0.500000000000031,1.15784136876797E-14));
#118262=DIRECTION('ref_axis',(0.437325728122469,0.757470380565119,0.484752338920285));
#118263=DIRECTION('',(0.264962354696018,0.4589282604266,0.848044693619243));
#118264=DIRECTION('',(-0.500000000000004,-0.866025403784436,2.11225360334866E-16));
#118265=DIRECTION('',(0.264962092561706,0.458927806396624,-0.84804502122311));
#118266=DIRECTION('center_axis',(0.866025403784434,-0.500000000000007,-2.48108921422391E-14));
#118267=DIRECTION('ref_axis',(0.437324790476918,0.757468756515445,-0.48475572254205));
#118268=DIRECTION('',(0.500000000000004,0.866025403784436,-7.04084534449558E-17));
#118269=DIRECTION('',(0.250002506357508,0.433017043030766,0.866022509672731));
#118270=DIRECTION('center_axis',(-0.866025877200519,0.49999918001571,1.63998888615131E-6));
#118271=DIRECTION('ref_axis',(0.433036167837011,0.750040644542055,0.499918702270653));
#118272=DIRECTION('',(0.500000000000004,0.866025403784436,-7.04084534449558E-17));
#118273=DIRECTION('center_axis',(-0.866024930320553,0.500000820059919,1.64014405730139E-6));
#118274=DIRECTION('ref_axis',(0.433021642321843,0.750015485165317,-0.499969028333883));
#118275=DIRECTION('',(0.250002584648429,0.433017178634621,-0.866022419268935));
#118276=DIRECTION('',(0.500000000000004,0.866025403784436,-7.04084534449558E-17));
#118277=DIRECTION('center_axis',(0.866025403784436,-0.500000000000004,-1.2195101864901E-16));
#118278=DIRECTION('ref_axis',(2.11225360334866E-16,1.2195101864901E-16,
1.));
#118279=DIRECTION('center_axis',(-0.866025403784422,0.50000000000003,5.29299032305956E-14));
#118280=DIRECTION('ref_axis',(0.437324790468609,0.757468756501035,-0.484755722572063));
#118281=DIRECTION('',(-0.264962092561705,-0.458927806396619,0.848045021223113));
#118282=DIRECTION('',(0.500000000000004,0.866025403784436,-2.11225360334866E-16));
#118283=DIRECTION('',(-0.264962354696036,-0.458928260426624,-0.848044693619225));
#118284=DIRECTION('center_axis',(-0.866025403784439,0.5,2.46730482184633E-14));
#118285=DIRECTION('ref_axis',(0.437325728131445,0.757470380580693,0.484752338887851));
#118286=DIRECTION('',(-0.500000000000004,-0.866025403784436,7.04084534449558E-17));
#118287=DIRECTION('',(-0.25000258464842,-0.4330171786346,0.866022419268947));
#118288=DIRECTION('center_axis',(0.866025877310547,-0.499999179825134,1.64037039928712E-6));
#118289=DIRECTION('ref_axis',(0.43303621917957,0.750040733470476,-0.499918524375456));
#118290=DIRECTION('',(-0.500000000000004,-0.866025403784436,7.04084534449558E-17));
#118291=DIRECTION('center_axis',(0.866024930426266,-0.50000081987682,1.63977751491898E-6));
#118292=DIRECTION('ref_axis',(0.433021589219966,0.750015393190659,0.499969212298594));
#118293=DIRECTION('',(-0.250002506357472,-0.433017043030735,-0.866022509672757));
#118294=DIRECTION('',(-0.500000000000004,-0.866025403784436,7.04084534449558E-17));
#118295=DIRECTION('center_axis',(-2.23587008033243E-16,-1.13923270769252E-16,
-1.));
#118296=DIRECTION('ref_axis',(-1.,-1.7597119642318E-48,2.23587008033243E-16));
#118297=DIRECTION('',(-0.587785252292477,-0.809016994374945,2.23587008033243E-16));
#118298=DIRECTION('center_axis',(2.23587008033243E-16,1.13923270769252E-16,
1.));
#118299=DIRECTION('ref_axis',(-1.,-2.1582735598713E-13,2.23587008033267E-16));
#118300=DIRECTION('',(0.587785252292477,0.809016994374945,-2.23587008033243E-16));
#118301=DIRECTION('center_axis',(-2.23587008033243E-16,-1.13923270769252E-16,
-1.));
#118302=DIRECTION('ref_axis',(-1.,-1.31193432862153E-33,2.23587008033243E-16));
#118303=DIRECTION('center_axis',(0.809016994374945,-0.587785252292477,-1.13923270769252E-16));
#118304=DIRECTION('ref_axis',(2.23587008033243E-16,1.13923270769252E-16,
1.));
#118305=DIRECTION('center_axis',(0.809016994374929,-0.587785252292498,1.59892379496519E-14));
#118306=DIRECTION('ref_axis',(0.514107226876986,0.707607892257023,0.484752338920019));
#118307=DIRECTION('',(0.311481929006017,0.428718095637374,0.848044693619242));
#118308=DIRECTION('',(-0.587785252292477,-0.809016994374945,2.23587008033243E-16));
#118309=DIRECTION('',(0.31148162084865,0.428717671495116,-0.848045021223109));
#118310=DIRECTION('center_axis',(0.809016994374931,-0.587785252292496,-3.45974107094534E-14));
#118311=DIRECTION('ref_axis',(0.514106124608479,0.707606375114597,-0.484755722542015));
#118312=DIRECTION('',(0.587785252292477,0.809016994374945,-8.27701011433323E-17));
#118313=DIRECTION('',(0.293895572546184,0.4045125525591,0.866022509672741));
#118314=DIRECTION('center_axis',(-0.809017550909309,0.58778448628559,1.63998887651158E-6));
#118315=DIRECTION('ref_axis',(0.50906454636235,0.700667238249654,0.499918702271177));
#118316=DIRECTION('',(0.587785252292477,0.809016994374945,-8.27701011433323E-17));
#118317=DIRECTION('center_axis',(-0.809016437785106,0.587786018369617,1.64014417022043E-6));
#118318=DIRECTION('ref_axis',(0.509047470549715,0.70064373503006,-0.49996902833082));
#118319=DIRECTION('',(0.293895664582666,0.404512679236473,-0.866022419268949));
#118320=DIRECTION('',(0.587785252292477,0.809016994374945,-8.27701011433323E-17));
#118321=DIRECTION('center_axis',(0.809016994374945,-0.587785252292477,-1.13923270769252E-16));
#118322=DIRECTION('ref_axis',(2.23587008033243E-16,1.13923270769252E-16,
1.));
#118323=DIRECTION('center_axis',(-0.809016994374939,0.587785252292484,2.23298029254063E-14));
#118324=DIRECTION('ref_axis',(0.514106124597969,0.707606375100143,-0.484755722574261));
#118325=DIRECTION('',(-0.311481620848633,-0.428717671495124,0.848045021223112));
#118326=DIRECTION('',(0.587785252292477,0.809016994374945,-2.23587008033243E-16));
#118327=DIRECTION('',(-0.311481929006026,-0.428718095637378,-0.848044693619237));
#118328=DIRECTION('center_axis',(-0.80901699437497,0.587785252292442,5.77542301873549E-14));
#118329=DIRECTION('ref_axis',(0.514107226887194,0.707607892271115,0.484752338888621));
#118330=DIRECTION('',(-0.587785252292477,-0.809016994374945,8.27701011433323E-17));
#118331=DIRECTION('',(-0.293895664582688,-0.404512679236433,0.86602241926896));
#118332=DIRECTION('center_axis',(0.809017551038662,-0.587784486107549,1.64037043199266E-6));
#118333=DIRECTION('ref_axis',(0.50906460671898,0.700667321323834,-0.499918524376656));
#118334=DIRECTION('',(-0.587785252292477,-0.809016994374945,8.27701011433323E-17));
#118335=DIRECTION('center_axis',(0.809016437909387,-0.58778601819856,1.6397775619102E-6));
#118336=DIRECTION('ref_axis',(0.509047408123843,0.700643649108601,0.499969212298298));
#118337=DIRECTION('',(-0.293895572546212,-0.404512552559089,-0.866022509672736));
#118338=DIRECTION('',(-0.587785252292477,-0.809016994374945,8.27701011433323E-17));
#118339=DIRECTION('center_axis',(-2.35041809182736E-16,-1.04647355694969E-16,
-1.));
#118340=DIRECTION('ref_axis',(-1.,1.47166508017397E-49,2.35041809182736E-16));
#118341=DIRECTION('',(-0.669130606358862,-0.743144825477391,2.35041809182736E-16));
#118342=DIRECTION('center_axis',(2.35041809182736E-16,1.04647355694969E-16,
1.));
#118343=DIRECTION('ref_axis',(-1.,1.48821490844481E-33,2.35041809182736E-16));
#118344=DIRECTION('',(0.669130606358862,0.743144825477391,-2.35041809182736E-16));
#118345=DIRECTION('center_axis',(-2.35041809182736E-16,-1.04647355694969E-16,
-1.));
#118346=DIRECTION('ref_axis',(-1.,-6.39873354129293E-36,2.35041809182736E-16));
#118347=DIRECTION('center_axis',(0.743144825477391,-0.669130606358862,-1.04647355694969E-16));
#118348=DIRECTION('ref_axis',(2.35041809182736E-16,1.04647355694969E-16,
1.));
#118349=DIRECTION('center_axis',(0.743144825477429,-0.669130606358819,-1.06962488352839E-13));
#118350=DIRECTION('ref_axis',(0.585256059269864,0.649992703804717,0.484752338920137));
#118351=DIRECTION('',(0.354588842120037,0.393810805677316,0.848044693619242));
#118352=DIRECTION('',(-0.669130606358862,-0.743144825477391,2.35041809182736E-16));
#118353=DIRECTION('',(0.354588491315835,0.393810416069778,-0.848045021223112));
#118354=DIRECTION('center_axis',(0.743144825477371,-0.669130606358884,-3.94217508482234E-14));
#118355=DIRECTION('ref_axis',(0.585254804454904,0.649991310191511,-0.484755722542782));
#118356=DIRECTION('',(0.669130606358862,0.743144825477391,-9.42249022928252E-17));
#118357=DIRECTION('',(0.334568657340454,0.371576137911918,0.866022509672739));
#118358=DIRECTION('center_axis',(-0.743145459032553,0.66912990272189,1.63998899132442E-6));
#118359=DIRECTION('ref_axis',(0.579515507192058,0.64361717507423,0.499918702264078));
#118360=DIRECTION('',(0.669130606358862,0.743144825477391,-9.42249022928252E-17));
#118361=DIRECTION('center_axis',(-0.743144191859738,0.669131310059876,1.64014411444931E-6));
#118362=DIRECTION('ref_axis',(0.579496068164192,0.64359558551295,-0.499969028331242));
#118363=DIRECTION('',(0.33456876211414,0.371576254274883,-0.866022419268959));
#118364=DIRECTION('',(0.669130606358862,0.743144825477391,-9.42249022928252E-17));
#118365=DIRECTION('center_axis',(0.743144825477391,-0.669130606358862,-1.04647355694969E-16));
#118366=DIRECTION('ref_axis',(2.35041809182736E-16,1.04647355694969E-16,
1.));
#118367=DIRECTION('center_axis',(-0.743144825477379,0.669130606358875,2.06757434494493E-14));
#118368=DIRECTION('ref_axis',(0.585254804443977,0.649991310179378,-0.484755722572244));
#118369=DIRECTION('',(-0.354588491315839,-0.393810416069783,0.848045021223108));
#118370=DIRECTION('',(0.669130606358862,0.743144825477391,-2.35041809182736E-16));
#118371=DIRECTION('',(-0.354588842120062,-0.393810805677307,-0.848044693619236));
#118372=DIRECTION('center_axis',(-0.743144825477412,0.669130606358838,6.12001866424422E-14));
#118373=DIRECTION('ref_axis',(0.585256059281444,0.649992703817579,0.484752338888909));
#118374=DIRECTION('',(-0.669130606358862,-0.743144825477391,9.42249022928252E-17));
#118375=DIRECTION('',(-0.334568762114167,-0.371576254274909,0.866022419268937));
#118376=DIRECTION('center_axis',(0.743145459179755,-0.669129902558405,1.64037040565622E-6));
#118377=DIRECTION('ref_axis',(0.579515575899146,0.643617251381539,-0.499918524376076));
#118378=DIRECTION('',(-0.669130606358862,-0.743144825477391,9.42249022928252E-17));
#118379=DIRECTION('center_axis',(0.743144192001206,-0.669131309902762,1.63977762043609E-6));
#118380=DIRECTION('ref_axis',(0.579495997097348,0.643595506585619,0.499969212303069));
#118381=DIRECTION('',(-0.334568657340481,-0.371576137911908,-0.866022509672733));
#118382=DIRECTION('',(-0.669130606358862,-0.743144825477391,9.42249022928252E-17));
#118383=DIRECTION('center_axis',(-2.4546426258488E-16,-9.42249022928242E-17,
-1.));
#118384=DIRECTION('ref_axis',(-1.,-5.4163468893589E-49,2.4546426258488E-16));
#118385=DIRECTION('',(-0.743144825477398,-0.669130606358854,2.4546426258488E-16));
#118386=DIRECTION('center_axis',(2.4546426258488E-16,9.42249022928242E-17,
1.));
#118387=DIRECTION('ref_axis',(-1.,2.32204937581661E-33,2.4546426258488E-16));
#118388=DIRECTION('',(0.743144825477398,0.669130606358854,-2.4546426258488E-16));
#118389=DIRECTION('center_axis',(-2.4546426258488E-16,-9.42249022928242E-17,
-1.));
#118390=DIRECTION('ref_axis',(-1.,9.76293207909597E-34,2.4546426258488E-16));
#118391=DIRECTION('center_axis',(0.669130606358854,-0.743144825477398,-9.42249022928242E-17));
#118392=DIRECTION('ref_axis',(2.4546426258488E-16,9.42249022928242E-17,
1.));
#118393=DIRECTION('center_axis',(0.669130606358848,-0.743144825477403,8.54597200757256E-15));
#118394=DIRECTION('ref_axis',(0.649992703802778,0.5852560592681,0.484752338924866));
#118395=DIRECTION('',(0.393810805677326,0.354588842120041,0.848044693619236));
#118396=DIRECTION('',(-0.743144825477398,-0.669130606358854,2.4546426258488E-16));
#118397=DIRECTION('',(0.393810416069787,0.354588491315845,-0.848045021223104));
#118398=DIRECTION('center_axis',(0.669130606358885,-0.74314482547737,4.49352824353853E-14));
#118399=DIRECTION('ref_axis',(0.649991310191743,0.58525480445511,-0.484755722542222));
#118400=DIRECTION('',(0.743144825477398,0.669130606358854,-1.04647355694969E-16));
#118401=DIRECTION('',(0.37157613791195,0.334568657340486,0.866022509672713));
#118402=DIRECTION('center_axis',(-0.66913130999335,0.743144191919639,1.63998879715907E-6));
#118403=DIRECTION('ref_axis',(0.643617174849723,0.57951550743858,0.499918702267346));
#118404=DIRECTION('',(0.743144825477398,0.669130606358854,-1.04647355694969E-16));
#118405=DIRECTION('center_axis',(-0.669129902655549,0.743145459092287,1.64014392062814E-6));
#118406=DIRECTION('ref_axis',(0.643595585588892,0.579496068080419,-0.499969028330582));
#118407=DIRECTION('',(0.371576254274919,0.33456876211414,-0.866022419268943));
#118408=DIRECTION('',(0.743144825477398,0.669130606358854,-1.04647355694969E-16));
#118409=DIRECTION('center_axis',(0.669130606358854,-0.743144825477398,-9.42249022928242E-17));
#118410=DIRECTION('ref_axis',(2.4546426258488E-16,9.42249022928242E-17,
1.));
#118411=DIRECTION('center_axis',(-0.669130606358856,0.743144825477396,-2.31568326633855E-14));
#118412=DIRECTION('ref_axis',(0.64999131017826,0.585254804442939,-0.484755722574996));
#118413=DIRECTION('',(-0.393810416069767,-0.354588491315837,0.848045021223116));
#118414=DIRECTION('',(0.743144825477398,0.669130606358854,-2.4546426258488E-16));
#118415=DIRECTION('',(-0.393810805677306,-0.354588842120033,-0.848044693619249));
#118416=DIRECTION('center_axis',(-0.669130606358852,0.7431448254774,1.18540902055183E-14));
#118417=DIRECTION('ref_axis',(0.649992703818894,0.585256059282603,0.484752338885747));
#118418=DIRECTION('',(-0.743144825477398,-0.669130606358854,1.04647355694969E-16));
#118419=DIRECTION('',(-0.371576254274903,-0.334568762114161,0.866022419268941));
#118420=DIRECTION('center_axis',(0.669131310156939,-0.743144191772342,1.64037041409087E-6));
#118421=DIRECTION('ref_axis',(0.643617251158495,0.579515576147658,-0.499918524375154));
#118422=DIRECTION('',(-0.743144825477398,-0.669130606358854,1.04647355694969E-16));
#118423=DIRECTION('center_axis',(0.66912990281256,-0.743145458950915,1.63977762973069E-6));
#118424=DIRECTION('ref_axis',(0.643595506661403,0.579495997014118,0.499969212301983));
#118425=DIRECTION('',(-0.371576137911901,-0.334568657340439,-0.866022509672752));
#118426=DIRECTION('',(-0.743144825477398,-0.669130606358854,1.04647355694969E-16));
#118427=DIRECTION('center_axis',(-2.54740177659163E-16,-8.27701011433311E-17,
-1.));
#118428=DIRECTION('ref_axis',(-1.,8.43631949586388E-49,2.54740177659163E-16));
#118429=DIRECTION('',(-0.80901699437495,-0.587785252292469,2.54740177659163E-16));
#118430=DIRECTION('center_axis',(2.54740177659163E-16,8.27701011433311E-17,
1.));
#118431=DIRECTION('ref_axis',(-1.,1.4388490399142E-13,2.54740177659151E-16));
#118432=DIRECTION('',(0.80901699437495,0.587785252292469,-2.54740177659163E-16));
#118433=DIRECTION('center_axis',(-2.54740177659163E-16,-8.27701011433311E-17,
-1.));
#118434=DIRECTION('ref_axis',(-1.,1.62537491717908E-33,2.54740177659163E-16));
#118435=DIRECTION('center_axis',(0.587785252292469,-0.80901699437495,-8.27701011433311E-17));
#118436=DIRECTION('ref_axis',(2.54740177659163E-16,8.27701011433311E-17,
1.));
#118437=DIRECTION('center_axis',(0.587785252292449,-0.809016994374965,4.85190668817008E-14));
#118438=DIRECTION('ref_axis',(0.707607892255849,0.514107226876106,0.484752338922666));
#118439=DIRECTION('',(0.428718095637378,0.31148192900602,0.848044693619239));
#118440=DIRECTION('',(-0.80901699437495,-0.587785252292469,2.54740177659163E-16));
#118441=DIRECTION('',(0.428717671495124,0.311481620848633,-0.848045021223112));
#118442=DIRECTION('center_axis',(0.587785252292468,-0.809016994374951,1.7505462789247E-14));
#118443=DIRECTION('ref_axis',(0.707606375113376,0.514106124607565,-0.484755722544767));
#118444=DIRECTION('',(0.80901699437495,0.587785252292469,-1.13923270769253E-16));
#118445=DIRECTION('',(0.40451255255907,0.293895572546188,0.866022509672753));
#118446=DIRECTION('center_axis',(-0.587786018297218,0.809016437837708,1.63998882108571E-6));
#118447=DIRECTION('ref_axis',(0.700667238053761,0.509064546632194,0.499918702270952));
#118448=DIRECTION('',(0.80901699437495,0.587785252292469,-1.13923270769253E-16));
#118449=DIRECTION('center_axis',(-0.587784486213293,0.809017550961835,1.64014400187427E-6));
#118450=DIRECTION('ref_axis',(0.700643735095865,0.509047470457802,-0.499969028332185));
#118451=DIRECTION('',(0.404512679236439,0.293895664582703,-0.866022419268952));
#118452=DIRECTION('',(0.80901699437495,0.587785252292469,-1.13923270769253E-16));
#118453=DIRECTION('center_axis',(0.587785252292469,-0.80901699437495,-8.27701011433311E-17));
#118454=DIRECTION('ref_axis',(2.54740177659163E-16,8.27701011433311E-17,
1.));
#118455=DIRECTION('center_axis',(-0.587785252292455,0.809016994374961,5.2378550071936E-15));
#118456=DIRECTION('ref_axis',(0.707606375100509,0.514106124598213,-0.484755722573467));
#118457=DIRECTION('',(-0.428717671495138,-0.311481620848646,0.8480450212231));
#118458=DIRECTION('',(0.80901699437495,0.587785252292469,-2.54740177659163E-16));
#118459=DIRECTION('',(-0.428718095637388,-0.311481929006024,-0.848044693619232));
#118460=DIRECTION('center_axis',(-0.587785252292488,0.809016994374937,2.35703421528348E-14));
#118461=DIRECTION('ref_axis',(0.707607892272611,0.514107226888294,0.484752338885272));
#118462=DIRECTION('',(-0.80901699437495,-0.587785252292469,1.13923270769253E-16));
#118463=DIRECTION('',(-0.404512679236475,-0.293895664582703,0.866022419268936));
#118464=DIRECTION('center_axis',(0.587786018475335,-0.809016437708297,1.64037056436227E-6));
#118465=DIRECTION('ref_axis',(0.700667321128012,0.509064606989453,-0.499918524375691));
#118466=DIRECTION('',(-0.80901699437495,-0.587785252292469,1.13923270769253E-16));
#118467=DIRECTION('center_axis',(0.58778448638428,-0.809017550837606,1.63977760081284E-6));
#118468=DIRECTION('ref_axis',(0.70064364917268,0.509047408031267,0.499969212302758));
#118469=DIRECTION('',(-0.404512552559119,-0.293895572546208,-0.866022509672724));
#118470=DIRECTION('',(-0.80901699437495,-0.587785252292469,1.13923270769253E-16));
#118471=DIRECTION('center_axis',(-2.62767925538921E-16,-7.04084534449545E-17,
-1.));
#118472=DIRECTION('ref_axis',(-1.,-5.53924399605649E-49,2.62767925538921E-16));
#118473=DIRECTION('',(-0.866025403784441,-0.499999999999995,2.62767925538921E-16));
#118474=DIRECTION('center_axis',(2.62767925538921E-16,7.04084534449545E-17,
1.));
#118475=DIRECTION('ref_axis',(-1.,1.19904086659517E-13,2.62767925538913E-16));
#118476=DIRECTION('',(0.866025403784441,0.499999999999995,-2.62767925538921E-16));
#118477=DIRECTION('center_axis',(-2.62767925538921E-16,-7.04084534449545E-17,
-1.));
#118478=DIRECTION('ref_axis',(-1.,1.9478478000333E-33,2.62767925538921E-16));
#118479=DIRECTION('center_axis',(0.499999999999995,-0.866025403784442,-7.04084534449545E-17));
#118480=DIRECTION('ref_axis',(2.62767925538921E-16,7.04084534449546E-17,
1.));
#118481=DIRECTION('center_axis',(0.500000000000008,-0.866025403784434,-2.67406220882127E-14));
#118482=DIRECTION('ref_axis',(0.757470380562976,0.437325728121196,0.484752338924782));
#118483=DIRECTION('',(0.458928260426606,0.264962354696021,0.848044693619239));
#118484=DIRECTION('',(-0.866025403784442,-0.499999999999995,2.62767925538921E-16));
#118485=DIRECTION('',(0.458927806396636,0.264962092561693,-0.848045021223108));
#118486=DIRECTION('center_axis',(0.500000000000001,-0.866025403784438,-1.18540929124028E-14));
#118487=DIRECTION('ref_axis',(0.757468756514725,0.437324790476515,-0.484755722543538));
#118488=DIRECTION('',(0.866025403784442,0.499999999999995,-1.21951018649011E-16));
#118489=DIRECTION('',(0.433017043030755,0.250002506357484,0.866022509672744));
#118490=DIRECTION('center_axis',(-0.50000081998247,0.866024930365269,1.63998882177424E-6));
#118491=DIRECTION('ref_axis',(0.750040644378195,0.433036168127423,0.499918702264939));
#118492=DIRECTION('',(0.866025403784442,0.499999999999995,-1.21951018649011E-16));
#118493=DIRECTION('center_axis',(-0.499999179938243,0.866025877245244,1.64014413493299E-6));
#118494=DIRECTION('ref_axis',(0.750015485221644,0.433021642223838,-0.499969028334268));
#118495=DIRECTION('',(0.433017178634609,0.250002584648407,-0.866022419268947));
#118496=DIRECTION('',(0.866025403784442,0.499999999999995,-1.21951018649011E-16));
#118497=DIRECTION('center_axis',(0.499999999999995,-0.866025403784442,-7.04084534449545E-17));
#118498=DIRECTION('ref_axis',(2.62767925538921E-16,7.04084534449546E-17,
1.));
#118499=DIRECTION('center_axis',(-0.500000000000014,0.866025403784431,-5.23785500719396E-14));
#118500=DIRECTION('ref_axis',(0.757468756499955,0.437324790467967,-0.48475572257433));
#118501=DIRECTION('',(-0.458927806396646,-0.264962092561691,0.848045021223103));
#118502=DIRECTION('',(0.866025403784442,0.499999999999995,-2.62767925538921E-16));
#118503=DIRECTION('',(-0.458928260426595,-0.264962354696022,-0.848044693619245));
#118504=DIRECTION('center_axis',(-0.499999999999967,0.866025403784458,-3.87325505552417E-14));
#118505=DIRECTION('ref_axis',(0.757470380580733,0.437325728131438,0.484752338887795));
#118506=DIRECTION('',(-0.866025403784442,-0.499999999999995,1.21951018649011E-16));
#118507=DIRECTION('',(-0.433017178634596,-0.2500025846484,0.866022419268955));
#118508=DIRECTION('center_axis',(0.500000820173097,-0.866024930255209,1.64037045746811E-6));
#118509=DIRECTION('ref_axis',(0.750040733301865,0.433036219467805,-0.499918524378755));
#118510=DIRECTION('',(-0.866025403784442,-0.499999999999995,1.21951018649011E-16));
#118511=DIRECTION('center_axis',(0.499999180121334,-0.866025877139537,1.63977761957551E-6));
#118512=DIRECTION('ref_axis',(0.75001539324847,0.433021589123389,0.499969212295514));
#118513=DIRECTION('',(-0.433017043030764,-0.250002506357468,-0.866022509672744));
#118514=DIRECTION('',(-0.866025403784442,-0.499999999999995,1.21951018649011E-16));
#118515=DIRECTION('center_axis',(-2.6945955253847E-16,-5.7275395996719E-17,
-1.));
#118516=DIRECTION('ref_axis',(-1.,-2.59568075678046E-49,2.6945955253847E-16));
#118517=DIRECTION('',(-0.913545457642603,-0.406736643075795,2.6945955253847E-16));
#118518=DIRECTION('center_axis',(2.6945955253847E-16,5.7275395996719E-17,
1.));
#118519=DIRECTION('ref_axis',(-1.,-4.79616346638067E-14,2.69459552538472E-16));
#118520=DIRECTION('',(0.913545457642603,0.406736643075795,-2.6945955253847E-16));
#118521=DIRECTION('center_axis',(-2.6945955253847E-16,-5.7275395996719E-17,
-1.));
#118522=DIRECTION('ref_axis',(-1.,1.96778773707771E-33,2.6945955253847E-16));
#118523=DIRECTION('center_axis',(0.406736643075795,-0.913545457642603,-5.7275395996719E-17));
#118524=DIRECTION('ref_axis',(2.6945955253847E-16,5.72753959967189E-17,
1.));
#118525=DIRECTION('center_axis',(0.406736643075756,-0.913545457642621,7.60867185190295E-14));
#118526=DIRECTION('ref_axis',(0.799033864871858,0.355752797173889,0.484752338922563));
#118527=DIRECTION('',(0.484110311157687,0.215539797381032,0.84804469361924));
#118528=DIRECTION('',(-0.913545457642603,-0.406736643075795,2.6945955253847E-16));
#118529=DIRECTION('',(0.484109832214429,0.215539584141774,-0.848045021223112));
#118530=DIRECTION('center_axis',(0.406736643075805,-0.913545457642599,3.50109255784926E-14));
#118531=DIRECTION('ref_axis',(0.799032151708166,0.355752034424264,-0.484755722544475));
#118532=DIRECTION('',(0.913545457642603,0.406736643075795,-1.28642645648559E-16));
#118533=DIRECTION('',(0.45677730816434,0.203370360392759,0.866022509672733));
#118534=DIRECTION('center_axis',(-0.406737508052106,0.913545072528375,1.63998884122466E-6));
#118535=DIRECTION('ref_axis',(0.791196448438914,0.352263354741736,0.499918702274427));
#118536=DIRECTION('',(0.913545457642603,0.406736643075795,-1.28642645648559E-16));
#118537=DIRECTION('center_axis',(-0.406735778016346,0.913545842789921,1.64014402562863E-6));
#118538=DIRECTION('ref_axis',(0.791169908742041,0.352251538263013,-0.499969028333208));
#118539=DIRECTION('',(0.456777451208943,0.203370424080329,-0.866022419268952));
#118540=DIRECTION('',(0.913545457642603,0.406736643075795,-1.28642645648559E-16));
#118541=DIRECTION('center_axis',(0.406736643075795,-0.913545457642603,-5.7275395996719E-17));
#118542=DIRECTION('ref_axis',(2.6945955253847E-16,5.72753959967189E-17,
1.));
#118543=DIRECTION('center_axis',(-0.406736643075747,0.913545457642625,8.04975611631868E-14));
#118544=DIRECTION('ref_axis',(0.799032151693964,0.355752034417941,-0.484755722572524));
#118545=DIRECTION('',(-0.484109832214455,-0.215539584141767,0.848045021223099));
#118546=DIRECTION('',(0.913545457642603,0.406736643075795,-2.6945955253847E-16));
#118547=DIRECTION('',(-0.484110311157686,-0.215539797381038,-0.848044693619239));
#118548=DIRECTION('center_axis',(-0.406736643075831,0.913545457642587,3.95595801044615E-14));
#118549=DIRECTION('ref_axis',(0.799033864889901,0.355752797181941,0.484752338886912));
#118550=DIRECTION('',(-0.913545457642603,-0.406736643075795,1.28642645648559E-16));
#118551=DIRECTION('',(-0.45677745120895,-0.203370424080332,0.866022419268948));
#118552=DIRECTION('center_axis',(0.406737508253185,-0.913545072438848,1.6403704280331E-6));
#118553=DIRECTION('ref_axis',(0.791196542247288,0.352263396508196,-0.499918524378168));
#118554=DIRECTION('',(-0.913545457642603,-0.406736643075795,1.28642645648559E-16));
#118555=DIRECTION('center_axis',(0.406735778209537,-0.913545842703908,1.63977743556656E-6));
#118556=DIRECTION('ref_axis',(0.791169811719127,0.352251495065917,0.499969212300265));
#118557=DIRECTION('',(-0.456777308164345,-0.203370360392764,-0.866022509672729));
#118558=DIRECTION('',(-0.913545457642603,-0.406736643075795,1.28642645648559E-16));
#118559=DIRECTION('center_axis',(-2.74741743792088E-16,-4.35148173242961E-17,
-1.));
#118560=DIRECTION('ref_axis',(-1.,-6.81793207750932E-49,2.74741743792088E-16));
#118561=DIRECTION('',(-0.951056516295155,-0.309016994374942,2.74741743792088E-16));
#118562=DIRECTION('center_axis',(2.74741743792088E-16,4.35148173242961E-17,
1.));
#118563=DIRECTION('ref_axis',(-1.,-3.5527136788005E-14,2.7474174379209E-16));
#118564=DIRECTION('',(0.951056516295155,0.309016994374942,-2.74741743792088E-16));
#118565=DIRECTION('center_axis',(-2.74741743792088E-16,-4.35148173242961E-17,
-1.));
#118566=DIRECTION('ref_axis',(-1.,1.72487465929315E-33,2.74741743792088E-16));
#118567=DIRECTION('center_axis',(0.309016994374942,-0.951056516295155,-4.35148173242961E-17));
#118568=DIRECTION('ref_axis',(2.74741743792088E-16,4.35148173242962E-17,
1.));
#118569=DIRECTION('center_axis',(0.309016994374943,-0.951056516295155,-1.10270606549342E-14));
#118570=DIRECTION('ref_axis',(0.831842966946887,0.270282164133852,0.484752338923827));
#118571=DIRECTION('',(0.50398834801313,0.163755740941354,0.848044693619236));
#118572=DIRECTION('',(-0.951056516295155,-0.309016994374942,2.74741743792088E-16));
#118573=DIRECTION('',(0.503987849404007,0.163755578933419,-0.84804502122311));
#118574=DIRECTION('center_axis',(0.309016994374941,-0.951056516295156,7.16759106331303E-15));
#118575=DIRECTION('ref_axis',(0.831841183439701,0.270281584637239,-0.48475572254448));
#118576=DIRECTION('',(0.951056516295155,0.309016994374942,-1.33924836902178E-16));
#118577=DIRECTION('',(0.475533025522861,0.154510046201606,0.866022509672729));
#118578=DIRECTION('center_axis',(-0.309017894868253,0.951056223705257,1.63998893959849E-6));
#118579=DIRECTION('ref_axis',(0.823683738646395,0.267631070328247,0.499918702275135));
#118580=DIRECTION('',(0.951056516295155,0.309016994374942,-1.33924836902178E-16));
#118581=DIRECTION('center_axis',(-0.309016093795537,0.951056808909256,1.64014401168567E-6));
#118582=DIRECTION('ref_axis',(0.823656109179299,0.267622092735483,-0.499969028332256));
#118583=DIRECTION('',(0.475533174441019,0.15451009458806,-0.866022419268945));
#118584=DIRECTION('',(0.951056516295155,0.309016994374942,-1.33924836902178E-16));
#118585=DIRECTION('center_axis',(0.309016994374942,-0.951056516295155,-4.35148173242961E-17));
#118586=DIRECTION('ref_axis',(2.74741743792088E-16,4.35148173242962E-17,
1.));
#118587=DIRECTION('center_axis',(-0.30901699437496,0.95105651629515,-3.73541764986754E-14));
#118588=DIRECTION('ref_axis',(0.831841183424385,0.270281584632265,-0.484755722573536));
#118589=DIRECTION('',(-0.50398784940401,-0.163755578933429,0.848045021223106));
#118590=DIRECTION('',(0.951056516295155,0.309016994374942,-2.74741743792088E-16));
#118591=DIRECTION('',(-0.503988348013116,-0.16375574094134,-0.848044693619247));
#118592=DIRECTION('center_axis',(-0.30901699437493,0.951056516295159,-3.51487558419452E-14));
#118593=DIRECTION('ref_axis',(0.831842966965654,0.270282164139961,0.484752338888217));
#118594=DIRECTION('',(-0.951056516295155,-0.309016994374942,1.33924836902178E-16));
#118595=DIRECTION('',(-0.475533174441039,-0.154510094588055,0.866022419268935));
#118596=DIRECTION('center_axis',(0.309017895077549,-0.951056223637252,1.64037043259453E-6));
#118597=DIRECTION('ref_axis',(0.82368383630952,0.267631102061202,-0.49991852437366));
#118598=DIRECTION('',(-0.951056516295155,-0.309016994374942,1.33924836902178E-16));
#118599=DIRECTION('center_axis',(0.309016093996535,-0.951056808843949,1.63977760201822E-6));
#118600=DIRECTION('ref_axis',(0.823656008170397,0.267622059915953,0.499969212303267));
#118601=DIRECTION('',(-0.475533025522838,-0.154510046201608,-0.866022509672741));
#118602=DIRECTION('',(-0.951056516295155,-0.309016994374942,1.33924836902178E-16));
#118603=DIRECTION('center_axis',(-2.78556626507032E-16,-2.92774812072074E-17,
-1.));
#118604=DIRECTION('ref_axis',(-1.,-3.4710284701162E-49,2.78556626507032E-16));
#118605=DIRECTION('',(-0.978147600733807,-0.207911690817753,2.78556626507032E-16));
#118606=DIRECTION('center_axis',(2.78556626507032E-16,2.92774812072074E-17,
1.));
#118607=DIRECTION('ref_axis',(-1.,-1.15463194561016E-14,2.78556626507033E-16));
#118608=DIRECTION('',(0.978147600733807,0.207911690817753,-2.78556626507032E-16));
#118609=DIRECTION('center_axis',(-2.78556626507032E-16,-2.92774812072074E-17,
-1.));
#118610=DIRECTION('ref_axis',(-1.,1.27221405500122E-33,2.78556626507032E-16));
#118611=DIRECTION('center_axis',(0.207911690817753,-0.978147600733807,-2.92774812072074E-17));
#118612=DIRECTION('ref_axis',(2.78556626507032E-16,2.92774812072074E-17,
1.));
#118613=DIRECTION('center_axis',(0.207911690817736,-0.978147600733811,3.70784914522103E-14));
#118614=DIRECTION('ref_axis',(0.855538223403387,0.1818502631439,0.484752338921918));
#118615=DIRECTION('',(0.518344583061388,0.11017754233581,0.848044693619243));
#118616=DIRECTION('',(-0.978147600733807,-0.207911690817753,2.78556626507032E-16));
#118617=DIRECTION('',(0.51834407024927,0.110177433334225,-0.848045021223109));
#118618=DIRECTION('center_axis',(0.207911690817736,-0.978147600733811,-2.73609005013009E-14));
#118619=DIRECTION('ref_axis',(0.855536389091131,0.181849873248789,-0.484755722545189));
#118620=DIRECTION('',(0.978147600733807,0.207911690817753,-1.37739719617122E-16));
#118621=DIRECTION('',(0.489078703542109,0.103956887610931,0.866022509672709));
#118622=DIRECTION('center_axis',(-0.207912616962004,0.978147403873936,1.63998883769561E-6));
#118623=DIRECTION('ref_axis',(0.847146577450102,0.180066563903761,0.499918702269151));
#118624=DIRECTION('',(0.978147600733807,0.207911690817753,-1.37739719617122E-16));
#118625=DIRECTION('center_axis',(-0.207910764585298,0.97814779760876,1.64014406599374E-6));
#118626=DIRECTION('ref_axis',(0.847118160922528,0.180060523556151,-0.499969028332675));
#118627=DIRECTION('',(0.48907885670219,0.103956920166115,-0.866022419268956));
#118628=DIRECTION('',(0.978147600733807,0.207911690817753,-1.37739719617122E-16));
#118629=DIRECTION('center_axis',(0.207911690817753,-0.978147600733807,-2.92774812072074E-17));
#118630=DIRECTION('ref_axis',(2.78556626507032E-16,2.92774812072074E-17,
1.));
#118631=DIRECTION('center_axis',(-0.207911690817752,0.978147600733807,-2.75676579326004E-15));
#118632=DIRECTION('ref_axis',(0.855536389076247,0.181849873245626,-0.484755722572644));
#118633=DIRECTION('',(-0.51834407024927,-0.110177433334225,0.848045021223109));
#118634=DIRECTION('',(0.978147600733807,0.207911690817753,-2.78556626507032E-16));
#118635=DIRECTION('',(-0.518344583061404,-0.110177542335807,-0.848044693619234));
#118636=DIRECTION('center_axis',(-0.20791169081776,0.978147600733806,7.09867029749066E-15));
#118637=DIRECTION('ref_axis',(0.855538223422756,0.181850263148017,0.484752338886189));
#118638=DIRECTION('',(-0.978147600733807,-0.207911690817753,1.37739719617122E-16));
#118639=DIRECTION('',(-0.489078856702205,-0.103956920166127,0.866022419268946));
#118640=DIRECTION('center_axis',(0.207912617177324,-0.978147403828168,1.64037046383705E-6));
#118641=DIRECTION('ref_axis',(0.84714667788957,0.180066585253091,-0.49991852437768));
#118642=DIRECTION('',(-0.978147600733807,-0.207911690817753,1.37739719617122E-16));
#118643=DIRECTION('center_axis',(0.207910764792092,-0.978147797564805,1.6397775222343E-6));
#118644=DIRECTION('ref_axis',(0.84711805703836,0.180060501475129,0.499969212300196));
#118645=DIRECTION('',(-0.489078703542019,-0.103956887610927,-0.866022509672761));
#118646=DIRECTION('',(-0.978147600733807,-0.207911690817753,1.37739719617122E-16));
#118647=DIRECTION('center_axis',(-2.80862404029962E-16,-1.47193748793057E-17,
-1.));
#118648=DIRECTION('ref_axis',(-1.,-1.64025481450153E-49,2.80862404029962E-16));
#118649=DIRECTION('',(-0.994521895368274,-0.104528463267647,2.80862404029962E-16));
#118650=DIRECTION('center_axis',(2.80862404029962E-16,1.47193748793057E-17,
1.));
#118651=DIRECTION('ref_axis',(-1.,-2.66453525910038E-15,2.80862404029962E-16));
#118652=DIRECTION('',(0.994521895368274,0.104528463267647,-2.80862404029962E-16));
#118653=DIRECTION('center_axis',(-2.80862404029962E-16,-1.47193748793057E-17,
-1.));
#118654=DIRECTION('ref_axis',(-1.,6.73550486588661E-34,2.80862404029962E-16));
#118655=DIRECTION('center_axis',(0.104528463267647,-0.994521895368274,-1.47193748793057E-17));
#118656=DIRECTION('ref_axis',(2.80862404029962E-16,1.47193748793057E-17,
1.));
#118657=DIRECTION('center_axis',(0.104528463267645,-0.994521895368274,4.75541990743991E-15));
#118658=DIRECTION('ref_axis',(0.869860024050967,0.0914259726160544,0.484752338920876));
#118659=DIRECTION('',(0.527021726387054,0.0553922155203039,0.848044693619246));
#118660=DIRECTION('',(-0.994521895368274,-0.104528463267647,2.80862404029962E-16));
#118661=DIRECTION('',(0.527021204990425,0.0553921607193091,-0.848045021223099));
#118662=DIRECTION('center_axis',(0.104528463267658,-0.994521895368273,1.5816943740677E-14));
#118663=DIRECTION('ref_axis',(0.86985815903197,0.0914257765946603,-0.484755722544434));
#118664=DIRECTION('',(0.994521895368274,0.104528463267647,-1.40045497140052E-16));
#118665=DIRECTION('',(0.497265932938971,0.052264755605219,0.866022509672735));
#118666=DIRECTION('center_axis',(-0.104529404915867,0.994521796395255,1.6399888852479E-6));
#118667=DIRECTION('ref_axis',(0.861327901069651,0.0905292105225472,0.499918702271794));
#118668=DIRECTION('',(0.994521895368274,0.104528463267647,-1.40045497140052E-16));
#118669=DIRECTION('center_axis',(-0.104527521530161,0.994521994347069,1.64014404434785E-6));
#118670=DIRECTION('ref_axis',(0.861299008823205,0.0905261736006209,-0.499969028334151));
#118671=DIRECTION('',(0.497266088663028,0.052264771972486,-0.866022419268946));
#118672=DIRECTION('',(0.994521895368274,0.104528463267647,-1.40045497140052E-16));
#118673=DIRECTION('center_axis',(0.104528463267647,-0.994521895368274,-1.47193748793057E-17));
#118674=DIRECTION('ref_axis',(2.80862404029962E-16,1.47193748793057E-17,
1.));
#118675=DIRECTION('center_axis',(-0.104528463267646,0.994521895368274,2.06757434494494E-16));
#118676=DIRECTION('ref_axis',(0.869858159016553,0.0914257765930377,-0.484755722572404));
#118677=DIRECTION('',(-0.527021204990406,-0.0553921607193066,0.848045021223111));
#118678=DIRECTION('',(0.994521895368274,0.104528463267647,-2.80862404029962E-16));
#118679=DIRECTION('',(-0.527021726387066,-0.0553922155203067,-0.848044693619239));
#118680=DIRECTION('center_axis',(-0.104528463267645,0.994521895368274,-5.92704510275897E-15));
#118681=DIRECTION('ref_axis',(0.869860024069577,0.0914259726180108,0.484752338887112));
#118682=DIRECTION('',(-0.994521895368274,-0.104528463267647,1.40045497140052E-16));
#118683=DIRECTION('',(-0.497266088663036,-0.0522647719724824,0.866022419268942));
#118684=DIRECTION('center_axis',(0.104529405134733,-0.99452179637225,1.64037042377313E-6));
#118685=DIRECTION('ref_axis',(0.86132800319141,0.0905292212562273,-0.499918524378763));
#118686=DIRECTION('',(-0.994521895368274,-0.104528463267647,1.40045497140052E-16));
#118687=DIRECTION('center_axis',(0.104527521740379,-0.994521994324975,1.63977757288379E-6));
#118688=DIRECTION('ref_axis',(0.861298903204249,0.0905261624998609,0.499969212294324));
#118689=DIRECTION('',(-0.497265932938974,-0.0522647556052289,-0.866022509672732));
#118690=DIRECTION('',(-0.994521895368274,-0.104528463267647,1.40045497140052E-16));
#118691=DIRECTION('center_axis',(-2.81633813779821E-16,0.,-1.));
#118692=DIRECTION('ref_axis',(-1.,0.,2.81633813779821E-16));
#118693=DIRECTION('',(-1.,0.,2.81633813779821E-16));
#118694=DIRECTION('',(1.,0.,-2.81633813779821E-16));
#118695=DIRECTION('center_axis',(0.,-1.,0.));
#118696=DIRECTION('ref_axis',(2.81633813779821E-16,0.,1.));
#118697=DIRECTION('center_axis',(0.,-1.,0.));
#118698=DIRECTION('ref_axis',(0.874651456242421,0.,0.484752338924746));
#118699=DIRECTION('',(0.529924709392058,0.,0.848044693619236));
#118700=DIRECTION('',(-1.,0.,2.81633813779821E-16));
#118701=DIRECTION('',(0.529924185123408,0.,-0.848045021223102));
#118702=DIRECTION('center_axis',(0.,-1.,0.));
#118703=DIRECTION('ref_axis',(0.874649580953487,0.,-0.484755722542694));
#118704=DIRECTION('',(1.,0.,-1.40816906889911E-16));
#118705=DIRECTION('',(0.500005012714997,0.,0.866022509672743));
#118706=DIRECTION('center_axis',(-9.46835258364187E-7,0.999999999998207,
1.6399888598465E-6));
#118707=DIRECTION('ref_axis',(0.866072335963656,1.66721433923257E-10,0.499918702269136));
#118708=DIRECTION('',(1.,0.,-1.40816906889911E-16));
#118709=DIRECTION('center_axis',(9.46924641656899E-7,0.999999999998207,
1.64014402974537E-6));
#118710=DIRECTION('ref_axis',(0.866043284545415,-5.65099970348825E-11,-0.499969028334545));
#118711=DIRECTION('',(0.500005169296866,0.,-0.866022419268931));
#118712=DIRECTION('',(1.,0.,-1.40816906889911E-16));
#118713=DIRECTION('center_axis',(0.,-1.,0.));
#118714=DIRECTION('ref_axis',(2.81633813779821E-16,0.,1.));
#118715=DIRECTION('center_axis',(0.,1.,0.));
#118716=DIRECTION('ref_axis',(0.87464958093593,0.,-0.484755722574372));
#118717=DIRECTION('',(-0.529924185123418,0.,0.848045021223096));
#118718=DIRECTION('',(1.,0.,-2.81633813779821E-16));
#118719=DIRECTION('',(-0.529924709392048,0.,-0.848044693619242));
#118720=DIRECTION('center_axis',(0.,1.,0.));
#118721=DIRECTION('ref_axis',(0.874651456262688,0.,0.484752338888178));
#118722=DIRECTION('',(-1.,0.,1.40816906889911E-16));
#118723=DIRECTION('',(-0.500005169296866,0.,0.866022419268931));
#118724=DIRECTION('center_axis',(9.47055351910275E-7,-0.999999999998206,
1.64037042964274E-6));
#118725=DIRECTION('ref_axis',(0.866072438647891,1.66973546088714E-10,-0.499918524376218));
#118726=DIRECTION('',(-1.,0.,1.40816906889911E-16));
#118727=DIRECTION('center_axis',(-9.46713274271685E-7,-0.999999999998207,
1.63977757417297E-6));
#118728=DIRECTION('ref_axis',(0.86604317834294,-5.62709268826161E-11,0.499969212297776));
#118729=DIRECTION('',(-0.500005012715,0.,-0.866022509672741));
#118730=DIRECTION('',(-1.,0.,1.40816906889911E-16));
#118731=DIRECTION('center_axis',(-2.80862404029962E-16,1.47193748793076E-17,
-1.));
#118732=DIRECTION('ref_axis',(-1.,7.08928067504585E-50,2.80862404029962E-16));
#118733=DIRECTION('',(-0.994521895368273,0.104528463267661,2.80862404029962E-16));
#118734=DIRECTION('center_axis',(2.80862404029962E-16,-1.47193748793076E-17,
1.));
#118735=DIRECTION('ref_axis',(-1.,2.29860575018392E-12,2.80862404029996E-16));
#118736=DIRECTION('',(0.994521895368273,-0.104528463267661,-2.80862404029962E-16));
#118737=DIRECTION('center_axis',(-2.80862404029962E-16,1.47193748793076E-17,
-1.));
#118738=DIRECTION('ref_axis',(-1.,-6.73550486588744E-34,2.80862404029962E-16));
#118739=DIRECTION('center_axis',(-0.104528463267661,-0.994521895368273,
1.47193748793076E-17));
#118740=DIRECTION('ref_axis',(2.80862404029962E-16,-1.47193748793076E-17,
1.));
#118741=DIRECTION('center_axis',(-0.104528463267661,-0.994521895368273,
6.20272161839949E-15));
#118742=DIRECTION('ref_axis',(0.869860024050468,-0.091425972616011,0.484752338921779));
#118743=DIRECTION('',(0.527021726387064,-0.0553922155203117,0.84804469361924));
#118744=DIRECTION('',(-0.994521895368273,0.104528463267661,2.80862404029962E-16));
#118745=DIRECTION('',(0.527021204990404,-0.0553921607193148,-0.848045021223112));
#118746=DIRECTION('center_axis',(-0.104528463267662,-0.994521895368273,
-2.75676579358242E-16));
#118747=DIRECTION('ref_axis',(0.869858159031523,-0.0914257765946247,-0.484755722545241));
#118748=DIRECTION('',(0.994521895368273,-0.104528463267661,-1.40045497140051E-16));
#118749=DIRECTION('',(0.497265932938997,-0.0522647556052269,0.866022509672719));
#118750=DIRECTION('center_axis',(0.104527521619062,0.994521994337726,1.6399888905836E-6));
#118751=DIRECTION('ref_axis',(0.861327901106544,-0.0905292101911616,0.499918702268239));
#118752=DIRECTION('',(0.994521895368273,-0.104528463267661,-1.40045497140051E-16));
#118753=DIRECTION('center_axis',(0.104529405004776,0.99452179638591,1.64014405953898E-6));
#118754=DIRECTION('ref_axis',(0.861299008813205,-0.0905261737132212,-0.499969028330989));
#118755=DIRECTION('',(0.497266088663028,-0.0522647719724816,-0.866022419268946));
#118756=DIRECTION('',(0.994521895368273,-0.104528463267661,-1.40045497140051E-16));
#118757=DIRECTION('center_axis',(-0.104528463267661,-0.994521895368273,
1.47193748793076E-17));
#118758=DIRECTION('ref_axis',(2.80862404029962E-16,-1.47193748793076E-17,
1.));
#118759=DIRECTION('center_axis',(0.104528463267664,0.994521895368272,1.32324758076483E-14));
#118760=DIRECTION('ref_axis',(0.869858159015868,-0.0914257765929747,-0.484755722573645));
#118761=DIRECTION('',(-0.527021204990425,0.055392160719319,0.848045021223099));
#118762=DIRECTION('',(0.994521895368273,-0.104528463267661,-2.80862404029962E-16));
#118763=DIRECTION('',(-0.52702172638706,0.0553922155203111,-0.848044693619242));
#118764=DIRECTION('center_axis',(0.104528463267665,0.994521895368272,-9.6142185097091E-15));
#118765=DIRECTION('ref_axis',(0.869860024069494,-0.0914259726180126,0.484752338887261));
#118766=DIRECTION('',(-0.994521895368273,0.104528463267661,1.40045497140051E-16));
#118767=DIRECTION('',(-0.497266088663009,0.0522647719724833,0.866022419268957));
#118768=DIRECTION('center_axis',(-0.104527521400192,-0.994521994360729,
1.64037043556414E-6));
#118769=DIRECTION('ref_axis',(0.8613280032289,-0.0905292209244034,-0.49991852437426));
#118770=DIRECTION('',(-0.994521895368273,0.104528463267661,1.40045497140051E-16));
#118771=DIRECTION('center_axis',(-0.104529404794561,-0.994521796408005,
1.63977758411581E-6));
#118772=DIRECTION('ref_axis',(0.861298903190469,-0.090526162611589,0.499969212297833));
#118773=DIRECTION('',(-0.497265932938974,0.0522647556052289,-0.866022509672732));
#118774=DIRECTION('',(-0.994521895368273,0.104528463267661,1.40045497140051E-16));
#118775=DIRECTION('center_axis',(-2.78556626507032E-16,2.92774812072093E-17,
-1.));
#118776=DIRECTION('ref_axis',(-1.,5.40378097023072E-49,2.78556626507032E-16));
#118777=DIRECTION('',(-0.978147600733804,0.207911690817766,2.78556626507032E-16));
#118778=DIRECTION('center_axis',(2.78556626507032E-16,-2.92774812072093E-17,
1.));
#118779=DIRECTION('ref_axis',(-1.,2.43272069155864E-12,2.78556626507103E-16));
#118780=DIRECTION('',(0.978147600733804,-0.207911690817766,-2.78556626507032E-16));
#118781=DIRECTION('center_axis',(-2.78556626507032E-16,2.92774812072093E-17,
-1.));
#118782=DIRECTION('ref_axis',(-1.,-1.27221405500129E-33,2.78556626507032E-16));
#118783=DIRECTION('center_axis',(-0.207911690817766,-0.978147600733804,
2.92774812072093E-17));
#118784=DIRECTION('ref_axis',(2.78556626507032E-16,-2.92774812072093E-17,
1.));
#118785=DIRECTION('center_axis',(-0.207911690817774,-0.978147600733803,
1.44730171095997E-14));
#118786=DIRECTION('ref_axis',(0.855538223402714,-0.181850263143766,0.484752338923156));
#118787=DIRECTION('',(0.518344583061382,-0.110177542335815,0.848044693619247));
#118788=DIRECTION('',(-0.978147600733804,0.207911690817766,2.78556626507032E-16));
#118789=DIRECTION('',(0.518344070249263,-0.110177433334233,-0.848045021223111));
#118790=DIRECTION('center_axis',(-0.207911690817754,-0.978147600733807,
2.06757434518653E-14));
#118791=DIRECTION('ref_axis',(0.855536389092462,-0.181849873249085,-0.484755722542728));
#118792=DIRECTION('',(0.978147600733804,-0.207911690817766,-1.37739719617121E-16));
#118793=DIRECTION('',(0.489078703542068,-0.103956887610929,0.866022509672733));
#118794=DIRECTION('center_axis',(0.207910764672729,0.978147797590176,1.63998893124938E-6));
#118795=DIRECTION('ref_axis',(0.847146577519436,-0.180066563577629,0.499918702269128));
#118796=DIRECTION('',(0.978147600733804,-0.207911690817766,-1.37739719617121E-16));
#118797=DIRECTION('center_axis',(0.207912617049499,0.978147403855338,1.64014410136726E-6));
#118798=DIRECTION('ref_axis',(0.847118160895452,-0.180060523665948,-0.499969028339007));
#118799=DIRECTION('',(0.489078856702189,-0.103956920166141,-0.866022419268953));
#118800=DIRECTION('',(0.978147600733804,-0.207911690817766,-1.37739719617121E-16));
#118801=DIRECTION('center_axis',(-0.207911690817766,-0.978147600733804,
2.92774812072093E-17));
#118802=DIRECTION('ref_axis',(2.78556626507032E-16,-2.92774812072093E-17,
1.));
#118803=DIRECTION('center_axis',(0.207911690817771,0.978147600733803,9.09732711775842E-15));
#118804=DIRECTION('ref_axis',(0.85553638907625,-0.18184987324564,-0.484755722572633));
#118805=DIRECTION('',(-0.518344070249254,0.110177433334231,0.848045021223118));
#118806=DIRECTION('',(0.978147600733804,-0.207911690817766,-2.78556626507032E-16));
#118807=DIRECTION('',(-0.518344583061409,0.110177542335818,-0.84804469361923));
#118808=DIRECTION('center_axis',(0.20791169081778,0.978147600733801,-1.84014074701936E-14));
#118809=DIRECTION('ref_axis',(0.855538223422332,-0.18185026314794,0.484752338886967));
#118810=DIRECTION('',(-0.978147600733804,0.207911690817766,1.37739719617121E-16));
#118811=DIRECTION('',(-0.489078856702197,0.103956920166125,0.86602241926895));
#118812=DIRECTION('center_axis',(-0.207910764457494,-0.978147797635925,
1.64037038904585E-6));
#118813=DIRECTION('ref_axis',(0.847146677957487,-0.180066584926125,-0.499918524380359));
#118814=DIRECTION('',(-0.978147600733804,0.207911690817766,1.37739719617121E-16));
#118815=DIRECTION('center_axis',(-0.207912616842688,-0.978147403899298,
1.63977753411228E-6));
#118816=DIRECTION('ref_axis',(0.847118057017983,-0.180060501585866,0.499969212294841));
#118817=DIRECTION('',(-0.489078703542045,0.103956887610933,-0.866022509672745));
#118818=DIRECTION('',(-0.978147600733804,0.207911690817766,1.37739719617121E-16));
#118819=DIRECTION('center_axis',(-2.74741743792087E-16,4.3514817324298E-17,
-1.));
#118820=DIRECTION('ref_axis',(-1.,-3.66113503437316E-49,2.74741743792087E-16));
#118821=DIRECTION('',(-0.951056516295151,0.309016994374954,2.74741743792088E-16));
#118822=DIRECTION('center_axis',(2.74741743792087E-16,-4.3514817324298E-17,
1.));
#118823=DIRECTION('ref_axis',(-1.,2.73292499741728E-12,2.74741743792206E-16));
#118824=DIRECTION('',(0.951056516295151,-0.309016994374954,-2.74741743792088E-16));
#118825=DIRECTION('center_axis',(-2.74741743792087E-16,4.3514817324298E-17,
-1.));
#118826=DIRECTION('ref_axis',(-1.,-1.72487465929319E-33,2.74741743792087E-16));
#118827=DIRECTION('center_axis',(-0.309016994374955,-0.951056516295151,
4.3514817324298E-17));
#118828=DIRECTION('ref_axis',(2.74741743792087E-16,-4.3514817324298E-17,
1.));
#118829=DIRECTION('center_axis',(-0.309016994374931,-0.951056516295159,
-5.10001555290581E-14));
#118830=DIRECTION('ref_axis',(0.831842966947536,-0.270282164134083,0.484752338922586));
#118831=DIRECTION('',(0.50398834801313,-0.163755740941351,0.848044693619237));
#118832=DIRECTION('',(-0.951056516295151,0.309016994374955,2.74741743792087E-16));
#118833=DIRECTION('',(0.50398784940401,-0.163755578933432,-0.848045021223106));
#118834=DIRECTION('center_axis',(-0.309016994374948,-0.951056516295153,
1.61270798924553E-14));
#118835=DIRECTION('ref_axis',(0.83184118344023,-0.27028158463743,-0.484755722543466));
#118836=DIRECTION('',(0.951056516295151,-0.309016994374955,-1.33924836902177E-16));
#118837=DIRECTION('',(0.475533025522889,-0.154510046201595,0.866022509672715));
#118838=DIRECTION('center_axis',(0.30901609388058,0.951056808881625,1.63998881953568E-6));
#118839=DIRECTION('ref_axis',(0.823683738751792,-0.267631070011922,0.499918702270823));
#118840=DIRECTION('',(0.951056516295151,-0.309016994374955,-1.33924836902177E-16));
#118841=DIRECTION('center_axis',(0.309017894953228,0.951056223677647,1.64014400566146E-6));
#118842=DIRECTION('ref_axis',(0.823656109143692,-0.267622092842761,-0.499969028333491));
#118843=DIRECTION('',(0.475533174441011,-0.154510094588075,-0.866022419268947));
#118844=DIRECTION('',(0.951056516295151,-0.309016994374955,-1.33924836902177E-16));
#118845=DIRECTION('center_axis',(-0.309016994374955,-0.951056516295151,
4.3514817324298E-17));
#118846=DIRECTION('ref_axis',(2.74741743792087E-16,-4.3514817324298E-17,
1.));
#118847=DIRECTION('center_axis',(0.309016994374951,0.951056516295153,1.18540929110179E-14));
#118848=DIRECTION('ref_axis',(0.831841183424048,-0.27028158463216,-0.484755722574172));
#118849=DIRECTION('',(-0.503987849403999,0.16375557893344,0.848045021223111));
#118850=DIRECTION('',(0.951056516295151,-0.309016994374955,-2.74741743792087E-16));
#118851=DIRECTION('',(-0.503988348013112,0.163755740941343,-0.848044693619249));
#118852=DIRECTION('center_axis',(0.309016994374947,0.951056516295154,3.17027993868513E-14));
#118853=DIRECTION('ref_axis',(0.831842966966367,-0.270282164140207,0.484752338886856));
#118854=DIRECTION('',(-0.951056516295151,0.309016994374955,1.33924836902177E-16));
#118855=DIRECTION('',(-0.475533174441046,0.154510094588057,0.86602241926893));
#118856=DIRECTION('center_axis',(-0.309016093671271,-0.951056808949632,
1.64037037088597E-6));
#118857=DIRECTION('ref_axis',(0.823683836409809,-0.267631101742673,-0.499918524378945));
#118858=DIRECTION('',(-0.951056516295151,0.309016994374955,1.33924836902177E-16));
#118859=DIRECTION('center_axis',(-0.309017894752234,-0.951056223742955,
1.63977758583762E-6));
#118860=DIRECTION('ref_axis',(0.82365600813909,-0.267622060024133,0.499969212296936));
#118861=DIRECTION('',(-0.475533025522828,0.154510046201581,-0.866022509672751));
#118862=DIRECTION('',(-0.951056516295151,0.309016994374955,1.33924836902177E-16));
#118863=DIRECTION('center_axis',(-2.69459552538469E-16,5.72753959967207E-17,
-1.));
#118864=DIRECTION('ref_axis',(-1.,-2.14642227784473E-49,2.69459552538469E-16));
#118865=DIRECTION('',(-0.913545457642598,0.406736643075807,2.69459552538469E-16));
#118866=DIRECTION('center_axis',(2.69459552538469E-16,-5.72753959967207E-17,
1.));
#118867=DIRECTION('ref_axis',(-1.,1.34203759216689E-12,2.69459552538546E-16));
#118868=DIRECTION('',(0.913545457642598,-0.406736643075807,-2.69459552538469E-16));
#118869=DIRECTION('center_axis',(-2.69459552538469E-16,5.72753959967207E-17,
-1.));
#118870=DIRECTION('ref_axis',(-1.,-1.96778773707772E-33,2.69459552538469E-16));
#118871=DIRECTION('center_axis',(-0.406736643075807,-0.913545457642598,
5.72753959967207E-17));
#118872=DIRECTION('ref_axis',(2.69459552538469E-16,-5.72753959967207E-17,
1.));
#118873=DIRECTION('center_axis',(-0.406736643075794,-0.913545457642604,
-3.39082115139216E-14));
#118874=DIRECTION('ref_axis',(0.79903386487193,-0.355752797173939,0.484752338922407));
#118875=DIRECTION('',(0.484110311157676,-0.215539797381039,0.848044693619245));
#118876=DIRECTION('',(-0.913545457642598,0.406736643075807,2.69459552538469E-16));
#118877=DIRECTION('',(0.484109832214419,-0.215539584141775,-0.848045021223117));
#118878=DIRECTION('center_axis',(-0.406736643075826,-0.913545457642589,
-5.91326262723355E-14));
#118879=DIRECTION('ref_axis',(0.799032151707498,-0.355752034423976,-0.484755722545787));
#118880=DIRECTION('',(0.913545457642598,-0.406736643075807,-1.28642645648558E-16));
#118881=DIRECTION('',(0.456777308164325,-0.20337036039277,0.866022509672739));
#118882=DIRECTION('center_axis',(0.406735778098031,0.913545842753553,1.63998883072505E-6));
#118883=DIRECTION('ref_axis',(0.791196448575512,-0.352263354437553,0.49991870227258));
#118884=DIRECTION('',(0.913545457642598,-0.406736643075807,-1.28642645648558E-16));
#118885=DIRECTION('center_axis',(0.406737508133729,0.913545072492033,1.64014393715232E-6));
#118886=DIRECTION('ref_axis',(0.791169908694848,-0.352251538365742,-0.499969028335509));
#118887=DIRECTION('',(0.456777451208943,-0.203370424080329,-0.866022419268952));
#118888=DIRECTION('',(0.913545457642598,-0.406736643075807,-1.28642645648558E-16));
#118889=DIRECTION('center_axis',(-0.406736643075807,-0.913545457642598,
5.72753959967207E-17));
#118890=DIRECTION('ref_axis',(2.69459552538469E-16,-5.72753959967207E-17,
1.));
#118891=DIRECTION('center_axis',(0.406736643075835,0.913545457642586,4.19028400575536E-14));
#118892=DIRECTION('ref_axis',(0.799032151693359,-0.355752034417699,-0.484755722573699));
#118893=DIRECTION('',(-0.484109832214429,0.215539584141774,0.848045021223112));
#118894=DIRECTION('',(0.913545457642598,-0.406736643075807,-2.69459552538469E-16));
#118895=DIRECTION('',(-0.484110311157675,0.215539797381046,-0.848044693619243));
#118896=DIRECTION('center_axis',(0.406736643075761,0.913545457642618,6.54731726467587E-14));
#118897=DIRECTION('ref_axis',(0.799033864888832,-0.355752797181447,0.484752338889038));
#118898=DIRECTION('',(-0.913545457642598,0.406736643075807,1.28642645648558E-16));
#118899=DIRECTION('',(-0.45677745120894,0.203370424080363,0.866022419268946));
#118900=DIRECTION('center_axis',(-0.406735777896922,-0.913545842843092,
1.6403704946483E-6));
#118901=DIRECTION('ref_axis',(0.791196542383054,-0.352263396203092,-0.499918524378287));
#118902=DIRECTION('',(-0.913545457642598,0.406736643075807,1.28642645648558E-16));
#118903=DIRECTION('center_axis',(-0.406737507940716,-0.913545072577969,
1.63977761028004E-6));
#118904=DIRECTION('ref_axis',(0.79116981167336,-0.352251495168743,0.499969212300243));
#118905=DIRECTION('',(-0.456777308164316,0.203370360392784,-0.86602250967274));
#118906=DIRECTION('',(-0.913545457642598,0.406736643075807,1.28642645648558E-16));
#118907=DIRECTION('center_axis',(-2.6276792553892E-16,7.04084534449562E-17,
-1.));
#118908=DIRECTION('ref_axis',(-1.,-1.29000548981482E-48,2.6276792553892E-16));
#118909=DIRECTION('',(-0.866025403784435,0.500000000000007,2.6276792553892E-16));
#118910=DIRECTION('center_axis',(2.6276792553892E-16,-7.04084534449562E-17,
1.));
#118911=DIRECTION('ref_axis',(-1.,-2.95344831741964E-33,2.6276792553892E-16));
#118912=DIRECTION('',(0.866025403784435,-0.500000000000007,-2.6276792553892E-16));
#118913=DIRECTION('center_axis',(-2.6276792553892E-16,7.04084534449562E-17,
-1.));
#118914=DIRECTION('ref_axis',(-1.,-1.94784780003327E-33,2.6276792553892E-16));
#118915=DIRECTION('center_axis',(-0.500000000000007,-0.866025403784435,
7.04084534449562E-17));
#118916=DIRECTION('ref_axis',(2.6276792553892E-16,-7.04084534449563E-17,
1.));
#118917=DIRECTION('center_axis',(-0.500000000000008,-0.866025403784434,
2.67406220882127E-14));
#118918=DIRECTION('ref_axis',(0.757470380563247,-0.437325728121353,0.484752338924217));
#118919=DIRECTION('',(0.458928260426606,-0.264962354696021,0.848044693619239));
#118920=DIRECTION('',(-0.866025403784435,0.500000000000007,2.6276792553892E-16));
#118921=DIRECTION('',(0.458927806396623,-0.264962092561713,-0.848045021223108));
#118922=DIRECTION('center_axis',(-0.49999999999998,-0.86602540378445,3.36325426817012E-14));
#118923=DIRECTION('ref_axis',(0.757468756514672,-0.437324790476473,-0.48475572254366));
#118924=DIRECTION('',(0.866025403784435,-0.500000000000007,-1.2195101864901E-16));
#118925=DIRECTION('',(0.433017043030766,-0.250002506357508,0.866022509672731));
#118926=DIRECTION('center_axis',(0.499999180015706,0.866025877200521,1.63998891403729E-6));
#118927=DIRECTION('ref_axis',(0.750040644540434,-0.433036167836086,0.499918702273888));
#118928=DIRECTION('',(0.866025403784435,-0.500000000000007,-1.2195101864901E-16));
#118929=DIRECTION('center_axis',(0.500000820059955,0.866024930320532,1.64014408707965E-6));
#118930=DIRECTION('ref_axis',(0.750015485168957,-0.43302164232397,-0.499969028326582));
#118931=DIRECTION('',(0.433017178634565,-0.25000258464842,-0.866022419268965));
#118932=DIRECTION('',(0.866025403784435,-0.500000000000007,-1.2195101864901E-16));
#118933=DIRECTION('center_axis',(-0.500000000000007,-0.866025403784435,
7.04084534449562E-17));
#118934=DIRECTION('ref_axis',(2.6276792553892E-16,-7.04084534449563E-17,
1.));
#118935=DIRECTION('center_axis',(0.499999999999996,0.866025403784441,-1.68162713388849E-14));
#118936=DIRECTION('ref_axis',(0.757468756500421,-0.437324790468254,-0.484755722573343));
#118937=DIRECTION('',(-0.458927806396634,0.264962092561705,0.848045021223105));
#118938=DIRECTION('',(0.866025403784435,-0.500000000000007,-2.6276792553892E-16));
#118939=DIRECTION('',(-0.458928260426591,0.264962354696021,-0.848044693619248));
#118940=DIRECTION('center_axis',(0.499999999999975,0.866025403784453,5.47217885068675E-14));
#118941=DIRECTION('ref_axis',(0.757470380580991,-0.437325728131605,0.48475233888724));
#118942=DIRECTION('',(-0.866025403784435,0.500000000000007,1.2195101864901E-16));
#118943=DIRECTION('',(-0.4330171786346,0.25000258464842,0.866022419268947));
#118944=DIRECTION('center_axis',(-0.499999179825081,-0.866025877310578,
1.64037050618159E-6));
#118945=DIRECTION('ref_axis',(0.750040733469961,-0.433036219179273,-0.499918524376487));
#118946=DIRECTION('',(-0.866025403784435,0.500000000000007,1.2195101864901E-16));
#118947=DIRECTION('center_axis',(-0.500000819876874,-0.866024930426235,
1.63977758687028E-6));
#118948=DIRECTION('ref_axis',(0.750015393191711,-0.433021589220595,0.499969212296472));
#118949=DIRECTION('',(-0.433017043030732,0.250002506357505,-0.866022509672749));
#118950=DIRECTION('',(-0.866025403784435,0.500000000000007,1.2195101864901E-16));
#118951=DIRECTION('center_axis',(-2.54740177659162E-16,8.27701011433327E-17,
-1.));
#118952=DIRECTION('ref_axis',(-1.,5.97523333326789E-49,2.54740177659162E-16));
#118953=DIRECTION('',(-0.809016994374943,0.58778525229248,2.54740177659162E-16));
#118954=DIRECTION('center_axis',(2.54740177659162E-16,-8.27701011433327E-17,
1.));
#118955=DIRECTION('ref_axis',(-1.,1.29496413592278E-12,2.54740177659269E-16));
#118956=DIRECTION('',(0.809016994374943,-0.58778525229248,-2.54740177659162E-16));
#118957=DIRECTION('center_axis',(-2.54740177659162E-16,8.27701011433327E-17,
-1.));
#118958=DIRECTION('ref_axis',(-1.,-1.62537491717902E-33,2.54740177659162E-16));
#118959=DIRECTION('center_axis',(-0.58778525229248,-0.809016994374943,8.27701011433327E-17));
#118960=DIRECTION('ref_axis',(2.54740177659162E-16,-8.27701011433327E-17,
1.));
#118961=DIRECTION('center_axis',(-0.587785252292429,-0.809016994374979,
-1.15232783844045E-13));
#118962=DIRECTION('ref_axis',(0.707607892254803,-0.51410722687536,0.484752338924985));
#118963=DIRECTION('',(0.428718095637373,-0.311481929006023,0.848044693619241));
#118964=DIRECTION('',(-0.809016994374943,0.58778525229248,2.54740177659162E-16));
#118965=DIRECTION('',(0.428717671495124,-0.311481620848633,-0.848045021223112));
#118966=DIRECTION('center_axis',(-0.58778525229247,-0.809016994374949,3.08757768881199E-14));
#118967=DIRECTION('ref_axis',(0.707606375113238,-0.514106124607496,-0.484755722545042));
#118968=DIRECTION('',(0.809016994374943,-0.58778525229248,-1.13923270769252E-16));
#118969=DIRECTION('',(0.404512552559091,-0.293895572546238,0.866022509672727));
#118970=DIRECTION('center_axis',(0.587784486285597,0.809017550909304,1.63998890801182E-6));
#118971=DIRECTION('ref_axis',(0.700667238252392,-0.509064546364368,0.499918702265284));
#118972=DIRECTION('',(0.809016994374943,-0.58778525229248,-1.13923270769252E-16));
#118973=DIRECTION('center_axis',(0.587786018369505,0.809016437785187,1.64014391821798E-6));
#118974=DIRECTION('ref_axis',(0.700643735029245,-0.50904747054913,-0.499969028332557));
#118975=DIRECTION('',(0.404512679236492,-0.29389566458268,-0.866022419268936));
#118976=DIRECTION('',(0.809016994374943,-0.58778525229248,-1.13923270769252E-16));
#118977=DIRECTION('center_axis',(-0.58778525229248,-0.809016994374943,8.27701011433327E-17));
#118978=DIRECTION('ref_axis',(2.54740177659162E-16,-8.27701011433327E-17,
1.));
#118979=DIRECTION('center_axis',(0.587785252292486,0.809016994374938,3.58379553123822E-15));
#118980=DIRECTION('ref_axis',(0.70760637510063,-0.514106124598336,-0.48475572257316));
#118981=DIRECTION('',(-0.428717671495123,0.311481620848639,0.84804502122311));
#118982=DIRECTION('',(0.809016994374943,-0.58778525229248,-2.54740177659162E-16));
#118983=DIRECTION('',(-0.428718095637372,0.311481929006025,-0.84804469361924));
#118984=DIRECTION('center_axis',(0.587785252292497,0.80901699437493,-3.52865941001464E-14));
#118985=DIRECTION('ref_axis',(0.707607892272525,-0.514107226888236,0.484752338885458));
#118986=DIRECTION('',(-0.809016994374943,0.58778525229248,1.13923270769252E-16));
#118987=DIRECTION('',(-0.404512679236479,0.293895664582671,0.866022419268945));
#118988=DIRECTION('center_axis',(-0.587784486107549,-0.809017551038662,
1.64037043199241E-6));
#118989=DIRECTION('ref_axis',(0.700667321322997,-0.509064606718372,-0.499918524378449));
#118990=DIRECTION('',(-0.809016994374943,0.58778525229248,1.13923270769252E-16));
#118991=DIRECTION('center_axis',(-0.587786018198577,-0.809016437909375,
1.63977768068271E-6));
#118992=DIRECTION('ref_axis',(0.70064364911207,-0.509047408126312,0.499969212290924));
#118993=DIRECTION('',(-0.404512552559121,0.293895572546191,-0.866022509672728));
#118994=DIRECTION('',(-0.809016994374943,0.58778525229248,1.13923270769252E-16));
#118995=DIRECTION('center_axis',(-2.45464262584879E-16,9.42249022928256E-17,
-1.));
#118996=DIRECTION('ref_axis',(-1.,8.38955225566875E-49,2.45464262584879E-16));
#118997=DIRECTION('',(-0.743144825477389,0.669130606358864,2.45464262584879E-16));
#118998=DIRECTION('center_axis',(2.45464262584879E-16,-9.42249022928256E-17,
1.));
#118999=DIRECTION('ref_axis',(-1.,-7.62234719786647E-12,2.4546426258416E-16));
#119000=DIRECTION('',(0.743144825477389,-0.669130606358864,-2.45464262584879E-16));
#119001=DIRECTION('center_axis',(-2.45464262584879E-16,9.42249022928256E-17,
-1.));
#119002=DIRECTION('ref_axis',(-1.,-9.76293207909489E-34,2.45464262584879E-16));
#119003=DIRECTION('center_axis',(-0.669130606358865,-0.743144825477389,
9.42249022928256E-17));
#119004=DIRECTION('ref_axis',(2.45464262584879E-16,-9.42249022928256E-17,
1.));
#119005=DIRECTION('center_axis',(-0.669130606358877,-0.743144825477377,
4.76920373325794E-14));
#119006=DIRECTION('ref_axis',(0.649992703803605,-0.585256059268853,0.484752338922848));
#119007=DIRECTION('',(0.393810805677312,-0.35458884212006,0.848044693619234));
#119008=DIRECTION('',(-0.743144825477389,0.669130606358864,2.45464262584879E-16));
#119009=DIRECTION('',(0.393810416069776,-0.354588491315847,-0.848045021223108));
#119010=DIRECTION('center_axis',(-0.669130606358856,-0.743144825477396,
-2.75676579358212E-16));
#119011=DIRECTION('ref_axis',(0.649991310190513,-0.585254804453987,-0.484755722545227));
#119012=DIRECTION('',(0.743144825477389,-0.669130606358864,-1.04647355694968E-16));
#119013=DIRECTION('',(0.37157613791192,-0.334568657340491,0.866022509672724));
#119014=DIRECTION('center_axis',(0.669129902721955,0.743145459032495,1.63998880765904E-6));
#119015=DIRECTION('ref_axis',(0.64361717507148,-0.579515507189562,0.499918702270512));
#119016=DIRECTION('',(0.743144825477389,-0.669130606358864,-1.04647355694968E-16));
#119017=DIRECTION('center_axis',(0.669131310059846,0.743144191859766,1.64014407726852E-6));
#119018=DIRECTION('ref_axis',(0.643595585511056,-0.579496068162464,-0.499969028335681));
#119019=DIRECTION('',(0.371576254274848,-0.334568762114175,-0.86602241926896));
#119020=DIRECTION('',(0.743144825477389,-0.669130606358864,-1.04647355694968E-16));
#119021=DIRECTION('center_axis',(-0.669130606358865,-0.743144825477389,
9.42249022928256E-17));
#119022=DIRECTION('ref_axis',(2.45464262584879E-16,-9.42249022928256E-17,
1.));
#119023=DIRECTION('center_axis',(0.669130606358884,0.743144825477371,6.75407619348737E-14));
#119024=DIRECTION('ref_axis',(0.649991310179091,-0.585254804443703,-0.484755722572959));
#119025=DIRECTION('',(-0.393810416069765,0.354588491315848,0.848045021223112));
#119026=DIRECTION('',(0.743144825477389,-0.669130606358864,-2.45464262584879E-16));
#119027=DIRECTION('',(-0.393810805677311,0.354588842120039,-0.848044693619244));
#119028=DIRECTION('center_axis',(0.669130606358803,0.743144825477444,1.49140995376402E-13));
#119029=DIRECTION('ref_axis',(0.649992703817709,-0.585256059281564,0.48475233888859));
#119030=DIRECTION('',(-0.743144825477389,0.669130606358864,1.04647355694968E-16));
#119031=DIRECTION('',(-0.371576254274903,0.334568762114161,0.866022419268941));
#119032=DIRECTION('center_axis',(-0.669129902558327,-0.743145459179825,
1.64037054921456E-6));
#119033=DIRECTION('ref_axis',(0.643617251381923,-0.579515575899465,-0.499918524375213));
#119034=DIRECTION('',(-0.743144825477389,0.669130606358864,1.04647355694968E-16));
#119035=DIRECTION('center_axis',(-0.669131309902758,-0.743144192001209,
1.63977761561624E-6));
#119036=DIRECTION('ref_axis',(0.643595506588468,-0.579495997099911,0.499969212296431));
#119037=DIRECTION('',(-0.371576137911887,0.334568657340422,-0.866022509672765));
#119038=DIRECTION('',(-0.743144825477389,0.669130606358864,1.04647355694968E-16));
#119039=DIRECTION('center_axis',(-2.35041809182734E-16,1.0464735569497E-16,
-1.));
#119040=DIRECTION('ref_axis',(-1.,-8.2261945837542E-49,2.35041809182734E-16));
#119041=DIRECTION('',(-0.669130606358852,0.7431448254774,2.35041809182734E-16));
#119042=DIRECTION('center_axis',(2.35041809182734E-16,-1.0464735569497E-16,
1.));
#119043=DIRECTION('ref_axis',(-1.,3.73923114693753E-12,2.35041809183126E-16));
#119044=DIRECTION('',(0.669130606358852,-0.7431448254774,-2.35041809182734E-16));
#119045=DIRECTION('center_axis',(-2.35041809182734E-16,1.0464735569497E-16,
-1.));
#119046=DIRECTION('ref_axis',(-1.,6.39873354143184E-36,2.35041809182734E-16));
#119047=DIRECTION('center_axis',(-0.7431448254774,-0.669130606358852,1.0464735569497E-16));
#119048=DIRECTION('ref_axis',(2.35041809182734E-16,-1.0464735569497E-16,
1.));
#119049=DIRECTION('center_axis',(-0.743144825477404,-0.669130606358848,
1.40595023350398E-14));
#119050=DIRECTION('ref_axis',(0.585256059269162,-0.649992703803956,0.484752338922004));
#119051=DIRECTION('',(0.354588842120045,-0.393810805677304,0.848044693619245));
#119052=DIRECTION('',(-0.669130606358852,0.7431448254774,2.35041809182734E-16));
#119053=DIRECTION('',(0.354588491315847,-0.393810416069776,-0.848045021223108));
#119054=DIRECTION('center_axis',(-0.743144825477429,-0.66913060635882,-8.628676933912E-14));
#119055=DIRECTION('ref_axis',(0.585254804454475,-0.649991310191057,-0.484755722543908));
#119056=DIRECTION('',(0.669130606358852,-0.7431448254774,-9.42249022928238E-17));
#119057=DIRECTION('',(0.334568657340465,-0.37157613791193,0.86602250967273));
#119058=DIRECTION('center_axis',(0.743144191919539,0.669131309993462,1.63998908117698E-6));
#119059=DIRECTION('ref_axis',(0.579515507436183,-0.643617174847078,0.499918702273529));
#119060=DIRECTION('',(0.669130606358852,-0.7431448254774,-9.42249022928238E-17));
#119061=DIRECTION('center_axis',(0.743145459092382,0.669129902655443,1.64014420223656E-6));
#119062=DIRECTION('ref_axis',(0.579496068080972,-0.643595585589479,-0.499969028329185));
#119063=DIRECTION('',(0.334568762114161,-0.371576254274903,-0.866022419268941));
#119064=DIRECTION('',(0.669130606358852,-0.7431448254774,-9.42249022928238E-17));
#119065=DIRECTION('center_axis',(-0.7431448254774,-0.669130606358852,1.0464735569497E-16));
#119066=DIRECTION('ref_axis',(2.35041809182734E-16,-1.0464735569497E-16,
1.));
#119067=DIRECTION('center_axis',(0.743144825477371,0.669130606358884,-6.75407619348654E-14));
#119068=DIRECTION('ref_axis',(0.585254804442919,-0.649991310178221,-0.484755722575073));
#119069=DIRECTION('',(-0.354588491315845,0.393810416069787,0.848045021223104));
#119070=DIRECTION('',(0.669130606358852,-0.7431448254774,-2.35041809182734E-16));
#119071=DIRECTION('',(-0.354588842120022,0.393810805677308,-0.848044693619253));
#119072=DIRECTION('center_axis',(0.743144825477395,0.669130606358858,3.80433592642209E-14));
#119073=DIRECTION('ref_axis',(0.585256059281062,-0.649992703817192,0.484752338889889));
#119074=DIRECTION('',(-0.669130606358852,0.7431448254774,9.42249022928238E-17));
#119075=DIRECTION('',(-0.334568762114157,0.371576254274933,0.86602241926893));
#119076=DIRECTION('center_axis',(-0.743144191772411,-0.669131310156863,
1.64037026881083E-6));
#119077=DIRECTION('ref_axis',(0.57951557614673,-0.643617251157489,-0.499918524377524));
#119078=DIRECTION('',(-0.669130606358852,0.7431448254774,9.42249022928238E-17));
#119079=DIRECTION('center_axis',(-0.743145458950914,-0.669129902812561,
1.63977760012488E-6));
#119080=DIRECTION('ref_axis',(0.579495997013497,-0.643595506660734,0.499969212303564));
#119081=DIRECTION('',(-0.33456865734047,0.371576137911897,-0.866022509672742));
#119082=DIRECTION('',(-0.669130606358852,0.7431448254774,9.42249022928238E-17));
#119083=DIRECTION('center_axis',(-2.23587008033241E-16,1.13923270769253E-16,
-1.));
#119084=DIRECTION('ref_axis',(-1.,-9.24278289080685E-49,2.23587008033241E-16));
#119085=DIRECTION('',(-0.587785252292466,0.809016994374953,2.23587008033241E-16));
#119086=DIRECTION('center_axis',(2.23587008033241E-16,-1.13923270769253E-16,
1.));
#119087=DIRECTION('ref_axis',(-1.,1.22390986234677E-12,2.23587008033381E-16));
#119088=DIRECTION('',(0.587785252292466,-0.809016994374953,-2.23587008033241E-16));
#119089=DIRECTION('center_axis',(-2.23587008033241E-16,1.13923270769253E-16,
-1.));
#119090=DIRECTION('ref_axis',(-1.,1.31193432862173E-33,2.23587008033241E-16));
#119091=DIRECTION('center_axis',(-0.809016994374953,-0.587785252292466,
1.13923270769253E-16));
#119092=DIRECTION('ref_axis',(2.23587008033241E-16,-1.13923270769253E-16,
1.));
#119093=DIRECTION('center_axis',(-0.809016994374928,-0.5877852522925,-5.81677449547676E-14));
#119094=DIRECTION('ref_axis',(0.514107226876155,-0.707607892255909,0.484752338922526));
#119095=DIRECTION('',(0.311481929006022,-0.428718095637368,0.848044693619243));
#119096=DIRECTION('',(-0.587785252292466,0.809016994374953,2.23587008033241E-16));
#119097=DIRECTION('',(0.311481620848633,-0.428717671495124,-0.848045021223112));
#119098=DIRECTION('center_axis',(-0.809016994374957,-0.58778525229246,-2.37081858248063E-14));
#119099=DIRECTION('ref_axis',(0.514106124608047,-0.707606375114021,-0.484755722543313));
#119100=DIRECTION('',(0.587785252292466,-0.809016994374953,-8.27701011433307E-17));
#119101=DIRECTION('',(0.293895572546188,-0.40451255255907,0.866022509672753));
#119102=DIRECTION('center_axis',(0.809016437837667,0.587786018297274,1.63998894088962E-6));
#119103=DIRECTION('ref_axis',(0.509064546633985,-0.700667238056223,0.499918702265677));
#119104=DIRECTION('',(0.587785252292466,-0.809016994374953,-8.27701011433307E-17));
#119105=DIRECTION('center_axis',(0.809017550961879,0.587784486213233,1.64014416574423E-6));
#119106=DIRECTION('ref_axis',(0.509047470456718,-0.700643735094342,-0.499969028335422));
#119107=DIRECTION('',(0.293895664582671,-0.404512679236479,-0.866022419268945));
#119108=DIRECTION('',(0.587785252292466,-0.809016994374953,-8.27701011433307E-17));
#119109=DIRECTION('center_axis',(-0.809016994374953,-0.587785252292466,
1.13923270769253E-16));
#119110=DIRECTION('ref_axis',(2.23587008033241E-16,-1.13923270769253E-16,
1.));
#119111=DIRECTION('center_axis',(0.809016994374949,0.587785252292471,6.67137321968949E-14));
#119112=DIRECTION('ref_axis',(0.514106124598002,-0.70760637510014,-0.48475572257423));
#119113=DIRECTION('',(-0.311481620848613,0.428717671495137,0.848045021223112));
#119114=DIRECTION('',(0.587785252292466,-0.809016994374953,-2.23587008033241E-16));
#119115=DIRECTION('',(-0.311481929006029,0.428718095637372,-0.848044693619239));
#119116=DIRECTION('center_axis',(0.809016994374976,0.587785252292435,-6.72650700034043E-14));
#119117=DIRECTION('ref_axis',(0.514107226886512,-0.707607892270182,0.484752338890708));
#119118=DIRECTION('',(-0.587785252292466,0.809016994374953,8.27701011433307E-17));
#119119=DIRECTION('',(-0.293895664582653,0.40451267923649,0.866022419268946));
#119120=DIRECTION('center_axis',(-0.809016437708326,-0.587786018475295,
1.64037045092715E-6));
#119121=DIRECTION('ref_axis',(0.509064606988709,-0.700667321126964,-0.499918524377919));
#119122=DIRECTION('',(-0.587785252292466,0.809016994374953,8.27701011433307E-17));
#119123=DIRECTION('center_axis',(-0.809017550837631,-0.587784486384246,
1.63977765520619E-6));
#119124=DIRECTION('ref_axis',(0.509047408030807,-0.700643649172062,0.499969212304091));
#119125=DIRECTION('',(-0.293895572546191,0.404512552559121,-0.866022509672728));
#119126=DIRECTION('',(-0.587785252292466,0.809016994374953,8.27701011433307E-17));
#119127=DIRECTION('center_axis',(-2.11225360334865E-16,1.21951018649011E-16,
-1.));
#119128=DIRECTION('ref_axis',(-1.,1.27854015281794E-48,2.11225360334865E-16));
#119129=DIRECTION('',(-0.499999999999992,0.866025403784443,2.11225360334865E-16));
#119130=DIRECTION('center_axis',(2.11225360334865E-16,-1.21951018649011E-16,
1.));
#119131=DIRECTION('ref_axis',(-1.,2.39808173319034E-12,2.11225360335157E-16));
#119132=DIRECTION('',(0.499999999999992,-0.866025403784443,-2.11225360334865E-16));
#119133=DIRECTION('center_axis',(-2.11225360334865E-16,1.21951018649011E-16,
-1.));
#119134=DIRECTION('ref_axis',(-1.,2.91189697534881E-33,2.11225360334865E-16));
#119135=DIRECTION('center_axis',(-0.866025403784443,-0.499999999999992,
1.21951018649011E-16));
#119136=DIRECTION('ref_axis',(2.11225360334865E-16,-1.21951018649011E-16,
1.));
#119137=DIRECTION('center_axis',(-0.866025403784462,-0.49999999999996,5.32055676600482E-14));
#119138=DIRECTION('ref_axis',(0.437325728121712,-0.757470380563887,0.484752338922892));
#119139=DIRECTION('',(0.264962354696012,-0.458928260426601,0.848044693619245));
#119140=DIRECTION('',(-0.499999999999992,0.866025403784443,2.11225360334865E-16));
#119141=DIRECTION('',(0.264962092561693,-0.458927806396636,-0.848045021223108));
#119142=DIRECTION('center_axis',(-0.866025403784433,-0.500000000000009,
2.35703475351271E-14));
#119143=DIRECTION('ref_axis',(0.437324790476389,-0.757468756514523,-0.484755722543968));
#119144=DIRECTION('',(0.499999999999992,-0.866025403784443,-7.04084534449541E-17));
#119145=DIRECTION('',(0.250002506357496,-0.433017043030782,0.866022509672727));
#119146=DIRECTION('center_axis',(0.866024930365251,0.500000819982501,1.63998888959419E-6));
#119147=DIRECTION('ref_axis',(0.433036168125046,-0.750040644374085,0.499918702273163));
#119148=DIRECTION('',(0.499999999999992,-0.866025403784443,-7.04084534449541E-17));
#119149=DIRECTION('center_axis',(0.866025877245205,0.499999179938311,1.6401439968823E-6));
#119150=DIRECTION('ref_axis',(0.433021642224347,-0.750015485222529,-0.499969028332501));
#119151=DIRECTION('',(0.250002584648424,-0.433017178634642,-0.866022419268925));
#119152=DIRECTION('',(0.499999999999992,-0.866025403784443,-7.04084534449541E-17));
#119153=DIRECTION('center_axis',(-0.866025403784443,-0.499999999999992,
1.21951018649011E-16));
#119154=DIRECTION('ref_axis',(2.11225360334865E-16,-1.21951018649011E-16,
1.));
#119155=DIRECTION('center_axis',(0.866025403784414,0.500000000000044,-1.1413010384097E-13));
#119156=DIRECTION('ref_axis',(0.437324790468524,-0.75746875650092,-0.484755722572319));
#119157=DIRECTION('',(-0.264962092561688,0.458927806396626,0.848045021223114));
#119158=DIRECTION('',(0.499999999999992,-0.866025403784443,-2.11225360334865E-16));
#119159=DIRECTION('',(-0.264962354696018,0.4589282604266,-0.848044693619243));
#119160=DIRECTION('center_axis',(0.86602540378443,0.500000000000014,4.09379626865015E-14));
#119161=DIRECTION('ref_axis',(0.437325728131046,-0.757470380580035,0.484752338889239));
#119162=DIRECTION('',(-0.499999999999992,0.866025403784443,7.04084534449541E-17));
#119163=DIRECTION('',(-0.250002584648412,0.433017178634622,0.866022419268938));
#119164=DIRECTION('center_axis',(-0.866024930255216,-0.500000820173085,
1.64037040754986E-6));
#119165=DIRECTION('ref_axis',(0.433036219468253,-0.750040733302616,-0.49991852437724));
#119166=DIRECTION('',(-0.499999999999992,0.866025403784443,7.04084534449541E-17));
#119167=DIRECTION('center_axis',(-0.866025877139515,-0.499999180121372,
1.63977754297659E-6));
#119168=DIRECTION('ref_axis',(0.433021589122641,-0.750015393247174,0.499969212298108));
#119169=DIRECTION('',(-0.250002506357496,0.433017043030747,-0.866022509672744));
#119170=DIRECTION('',(-0.499999999999992,0.866025403784443,7.04084534449541E-17));
#119171=DIRECTION('center_axis',(-1.98092302886629E-16,1.28642645648559E-16,
-1.));
#119172=DIRECTION('ref_axis',(-1.,3.58748490176176E-52,1.98092302886629E-16));
#119173=DIRECTION('',(-0.406736643075792,0.913545457642605,1.98092302886629E-16));
#119174=DIRECTION('center_axis',(1.98092302886629E-16,-1.28642645648559E-16,
1.));
#119175=DIRECTION('ref_axis',(-1.,-7.04858393874019E-12,1.98092302885722E-16));
#119176=DIRECTION('',(0.406736643075792,-0.913545457642605,-1.98092302886629E-16));
#119177=DIRECTION('center_axis',(-1.98092302886629E-16,1.28642645648559E-16,
-1.));
#119178=DIRECTION('ref_axis',(-1.,4.76114818715962E-33,1.98092302886629E-16));
#119179=DIRECTION('center_axis',(-0.913545457642605,-0.406736643075792,
1.28642645648559E-16));
#119180=DIRECTION('ref_axis',(1.98092302886629E-16,-1.28642645648559E-16,
1.));
#119181=DIRECTION('center_axis',(-0.913545457642622,-0.406736643075753,
7.88434836827655E-14));
#119182=DIRECTION('ref_axis',(0.355752797173625,-0.799033864871266,0.484752338923733));
#119183=DIRECTION('',(0.215539797381043,-0.484110311157696,0.848044693619233));
#119184=DIRECTION('',(-0.406736643075792,0.913545457642605,1.98092302886629E-16));
#119185=DIRECTION('',(0.21553958414176,-0.48410983221444,-0.848045021223109));
#119186=DIRECTION('center_axis',(-0.91354545764262,-0.406736643075758,-4.30055463798799E-14));
#119187=DIRECTION('ref_axis',(0.355752034424546,-0.799032151708817,-0.484755722543195));
#119188=DIRECTION('',(0.406736643075792,-0.913545457642605,-5.72753959967185E-17));
#119189=DIRECTION('',(0.20337036039277,-0.456777308164325,0.866022509672739));
#119190=DIRECTION('center_axis',(0.913545072528382,0.40673750805209,1.63998879457736E-6));
#119191=DIRECTION('ref_axis',(0.352263354742908,-0.791196448441526,0.499918702269468));
#119192=DIRECTION('',(0.406736643075792,-0.913545457642605,-5.72753959967185E-17));
#119193=DIRECTION('center_axis',(0.91354584278993,0.406735778016327,1.6401441017111E-6));
#119194=DIRECTION('ref_axis',(0.352251538262862,-0.791169908741651,-0.499969028333931));
#119195=DIRECTION('',(0.203370424080329,-0.456777451208978,-0.866022419268934));
#119196=DIRECTION('',(0.406736643075792,-0.913545457642605,-5.72753959967185E-17));
#119197=DIRECTION('center_axis',(-0.913545457642605,-0.406736643075792,
1.28642645648559E-16));
#119198=DIRECTION('ref_axis',(1.98092302886629E-16,-1.28642645648559E-16,
1.));
#119199=DIRECTION('center_axis',(0.91354545764259,0.406736643075824,-5.29299032305855E-14));
#119200=DIRECTION('ref_axis',(0.35575203441816,-0.799032151694434,-0.484755722571589));
#119201=DIRECTION('',(-0.215539584141764,0.484109832214436,0.848045021223111));
#119202=DIRECTION('',(0.406736643075792,-0.913545457642605,-1.98092302886629E-16));
#119203=DIRECTION('',(-0.215539797381044,0.48411031115771,-0.848044693619224));
#119204=DIRECTION('center_axis',(0.913545457642615,0.406736643075768,-3.6802814940392E-14));
#119205=DIRECTION('ref_axis',(0.355752797182121,-0.799033864890364,0.484752338886018));
#119206=DIRECTION('',(-0.406736643075792,0.913545457642605,5.72753959967185E-17));
#119207=DIRECTION('',(-0.203370424080329,0.456777451208908,0.86602241926897));
#119208=DIRECTION('center_axis',(-0.913545072438882,-0.406737508253109,
1.64037028550778E-6));
#119209=DIRECTION('ref_axis',(0.352263396509503,-0.791196542250226,-0.499918524372597));
#119210=DIRECTION('',(-0.406736643075792,0.913545457642605,5.72753959967185E-17));
#119211=DIRECTION('center_axis',(-0.913545842703948,-0.406735778209447,
1.63977759031303E-6));
#119212=DIRECTION('ref_axis',(0.352251495066461,-0.791169811720368,0.499969212297917));
#119213=DIRECTION('',(-0.20337036039277,0.45677730816429,-0.866022509672757));
#119214=DIRECTION('',(-0.406736643075792,0.913545457642605,5.72753959967185E-17));
#119215=DIRECTION('center_axis',(-1.84331724214206E-16,1.33924836902178E-16,
-1.));
#119216=DIRECTION('ref_axis',(-1.,-8.60748644135896E-49,1.84331724214206E-16));
#119217=DIRECTION('',(-0.309016994374938,0.951056516295157,1.84331724214206E-16));
#119218=DIRECTION('center_axis',(1.84331724214206E-16,-1.33924836902178E-16,
1.));
#119219=DIRECTION('ref_axis',(-1.,-6.90292267790937E-12,1.84331724213282E-16));
#119220=DIRECTION('',(0.309016994374938,-0.951056516295157,-1.84331724214206E-16));
#119221=DIRECTION('center_axis',(-1.84331724214206E-16,1.33924836902178E-16,
-1.));
#119222=DIRECTION('ref_axis',(-1.,6.79952878369311E-33,1.84331724214206E-16));
#119223=DIRECTION('center_axis',(-0.951056516295157,-0.309016994374938,
1.33924836902178E-16));
#119224=DIRECTION('ref_axis',(1.84331724214206E-16,-1.33924836902178E-16,
1.));
#119225=DIRECTION('center_axis',(-0.95105651629516,-0.309016994374928,2.99109020265034E-14));
#119226=DIRECTION('ref_axis',(0.270282164134193,-0.831842966947917,0.484752338921869));
#119227=DIRECTION('',(0.163755740941343,-0.503988348013141,0.848044693619232));
#119228=DIRECTION('',(-0.309016994374938,0.951056516295157,1.84331724214206E-16));
#119229=DIRECTION('',(0.163755578933417,-0.503987849404001,-0.848045021223114));
#119230=DIRECTION('center_axis',(-0.951056516295151,-0.309016994374956,
2.37081858248069E-14));
#119231=DIRECTION('ref_axis',(0.270281584637447,-0.831841183440324,-0.484755722543294));
#119232=DIRECTION('',(0.309016994374938,-0.951056516295157,-4.35148173242957E-17));
#119233=DIRECTION('',(0.15451004620159,-0.475533025522892,0.866022509672715));
#119234=DIRECTION('center_axis',(0.951056223705273,0.309017894868205,1.6399888086916E-6));
#119235=DIRECTION('ref_axis',(0.267631070328562,-0.823683738647293,0.499918702273485));
#119236=DIRECTION('',(0.309016994374938,-0.951056516295157,-4.35148173242957E-17));
#119237=DIRECTION('center_axis',(0.951056808909271,0.309016093795493,1.6401440891452E-6));
#119238=DIRECTION('ref_axis',(0.267622092735315,-0.823656109178786,-0.49996902833319));
#119239=DIRECTION('',(0.154510094588032,-0.475533174441048,-0.866022419268934));
#119240=DIRECTION('',(0.309016994374938,-0.951056516295157,-4.35148173242957E-17));
#119241=DIRECTION('center_axis',(-0.951056516295157,-0.309016994374938,
1.33924836902178E-16));
#119242=DIRECTION('ref_axis',(1.84331724214206E-16,-1.33924836902178E-16,
1.));
#119243=DIRECTION('center_axis',(0.951056516295149,0.30901699437496,-5.03109757269963E-14));
#119244=DIRECTION('ref_axis',(0.270281584632175,-0.831841183424126,-0.48475572257403));
#119245=DIRECTION('',(-0.163755578933422,0.503987849404011,0.848045021223107));
#119246=DIRECTION('',(0.309016994374938,-0.951056516295157,-1.84331724214206E-16));
#119247=DIRECTION('',(-0.163755740941338,0.503988348013136,-0.848044693619236));
#119248=DIRECTION('center_axis',(0.951056516295152,0.309016994374954,2.77054898989464E-14));
#119249=DIRECTION('ref_axis',(0.270282164140366,-0.831842966966927,0.484752338885807));
#119250=DIRECTION('',(-0.309016994374938,0.951056516295157,4.35148173242957E-17));
#119251=DIRECTION('',(-0.154510094588047,0.475533174441005,0.866022419268955));
#119252=DIRECTION('center_axis',(-0.951056223637261,-0.309017895077522,
1.64037037174637E-6));
#119253=DIRECTION('ref_axis',(0.26763110206138,-0.823683836310049,-0.499918524372694));
#119254=DIRECTION('',(-0.309016994374938,0.951056516295157,4.35148173242957E-17));
#119255=DIRECTION('center_axis',(-0.951056808843949,-0.309016093996535,
1.63977763110796E-6));
#119256=DIRECTION('ref_axis',(0.267622059916075,-0.823656008170728,0.499969212302656));
#119257=DIRECTION('',(-0.154510046201584,0.475533025522848,-0.86602250967274));
#119258=DIRECTION('',(-0.309016994374938,0.951056516295157,4.35148173242957E-17));
#119259=DIRECTION('center_axis',(-1.70094388097117E-16,1.37739719617122E-16,
-1.));
#119260=DIRECTION('ref_axis',(-1.,-8.13991384035174E-49,1.70094388097117E-16));
#119261=DIRECTION('',(-0.207911690817749,0.978147600733808,1.70094388097117E-16));
#119262=DIRECTION('center_axis',(1.70094388097117E-16,-1.37739719617122E-16,
1.));
#119263=DIRECTION('ref_axis',(-1.,-9.01323460311687E-12,1.70094388095876E-16));
#119264=DIRECTION('',(0.207911690817749,-0.978147600733808,-1.70094388097117E-16));
#119265=DIRECTION('center_axis',(-1.70094388097117E-16,1.37739719617122E-16,
-1.));
#119266=DIRECTION('ref_axis',(-1.,-7.23724578308818E-33,1.70094388097117E-16));
#119267=DIRECTION('center_axis',(-0.978147600733808,-0.207911690817749,
1.37739719617122E-16));
#119268=DIRECTION('ref_axis',(1.70094388097117E-16,-1.37739719617122E-16,
1.));
#119269=DIRECTION('center_axis',(-0.978147600733812,-0.20791169081773,3.10136080919944E-14));
#119270=DIRECTION('ref_axis',(0.181850263143769,-0.855538223402807,0.484752338922991));
#119271=DIRECTION('',(0.110177542335806,-0.518344583061388,0.848044693619244));
#119272=DIRECTION('',(-0.207911690817749,0.978147600733808,1.70094388097117E-16));
#119273=DIRECTION('',(0.110177433334219,-0.518344070249257,-0.848045021223117));
#119274=DIRECTION('center_axis',(-0.978147600733808,-0.20791169081775,-1.72297862098883E-15));
#119275=DIRECTION('ref_axis',(0.181849873248976,-0.85553638909201,-0.484755722543567));
#119276=DIRECTION('',(0.207911690817749,-0.978147600733808,-2.92774812072069E-17));
#119277=DIRECTION('',(0.103956887610952,-0.489078703542055,0.866022509672737));
#119278=DIRECTION('center_axis',(0.978147403873943,0.207912616961972,1.63998880283903E-6));
#119279=DIRECTION('ref_axis',(0.180066563903965,-0.847146577451112,0.499918702267365));
#119280=DIRECTION('',(0.207911690817749,-0.978147600733808,-2.92774812072069E-17));
#119281=DIRECTION('center_axis',(0.978147797608769,0.207910764585256,1.64014411823538E-6));
#119282=DIRECTION('ref_axis',(0.180060523556428,-0.847118160923886,-0.499969028330273));
#119283=DIRECTION('',(0.103956920166112,-0.48907885670221,-0.866022419268945));
#119284=DIRECTION('',(0.207911690817749,-0.978147600733808,-2.92774812072069E-17));
#119285=DIRECTION('center_axis',(-0.978147600733808,-0.207911690817749,
1.37739719617122E-16));
#119286=DIRECTION('ref_axis',(1.70094388097117E-16,-1.37739719617122E-16,
1.));
#119287=DIRECTION('center_axis',(0.978147600733809,0.207911690817741,1.07513865937135E-14));
#119288=DIRECTION('ref_axis',(0.181849873245357,-0.855536389075001,-0.484755722574944));
#119289=DIRECTION('',(-0.110177433334221,0.518344070249267,0.848045021223111));
#119290=DIRECTION('',(0.207911690817749,-0.978147600733808,-1.70094388097117E-16));
#119291=DIRECTION('',(-0.110177542335799,0.518344583061388,-0.848044693619245));
#119292=DIRECTION('center_axis',(0.978147600733805,0.20791169081776,9.71759720336066E-15));
#119293=DIRECTION('ref_axis',(0.181850263147746,-0.855538223421482,0.48475233888854));
#119294=DIRECTION('',(-0.207911690817749,0.978147600733808,2.92774812072069E-17));
#119295=DIRECTION('',(-0.103956920166105,0.489078856702183,0.866022419268961));
#119296=DIRECTION('center_axis',(-0.978147403828172,-0.207912617177303,
1.64037044886142E-6));
#119297=DIRECTION('ref_axis',(0.180066585253005,-0.84714667788922,-0.499918524378303));
#119298=DIRECTION('',(-0.207911690817749,0.978147600733808,2.92774812072069E-17));
#119299=DIRECTION('center_axis',(-0.978147797564805,-0.207910764792092,
1.63977752223455E-6));
#119300=DIRECTION('ref_axis',(0.18006050147523,-0.847118057038833,0.499969212299358));
#119301=DIRECTION('',(-0.103956887610913,0.489078703542031,-0.866022509672756));
#119302=DIRECTION('',(-0.207911690817749,0.978147600733808,2.92774812072069E-17));
#119303=DIRECTION('center_axis',(-1.55536281769216E-16,1.40045497140052E-16,
-1.));
#119304=DIRECTION('ref_axis',(-1.,-1.27395445529282E-48,1.55536281769216E-16));
#119305=DIRECTION('',(-0.104528463267644,0.994521895368274,1.55536281769216E-16));
#119306=DIRECTION('center_axis',(1.55536281769216E-16,-1.40045497140052E-16,
1.));
#119307=DIRECTION('ref_axis',(-1.,2.20623519453511E-12,1.55536281769525E-16));
#119308=DIRECTION('',(0.104528463267644,-0.994521895368274,-1.55536281769216E-16));
#119309=DIRECTION('center_axis',(-1.55536281769216E-16,1.40045497140052E-16,
-1.));
#119310=DIRECTION('ref_axis',(-1.,-5.31960080738386E-33,1.55536281769216E-16));
#119311=DIRECTION('center_axis',(-0.994521895368274,-0.104528463267644,
1.40045497140052E-16));
#119312=DIRECTION('ref_axis',(1.55536281769216E-16,-1.40045497140052E-16,
1.));
#119313=DIRECTION('center_axis',(-0.994521895368274,-0.104528463267649,
-1.28189580113589E-14));
#119314=DIRECTION('ref_axis',(0.091425972615971,-0.869860024050217,0.484752338922238));
#119315=DIRECTION('',(0.0553922155203038,-0.527021726387067,0.848044693619238));
#119316=DIRECTION('',(-0.104528463267644,0.994521895368274,1.55536281769216E-16));
#119317=DIRECTION('',(0.0553921607193063,-0.527021204990403,-0.848045021223113));
#119318=DIRECTION('center_axis',(-0.994521895368274,-0.104528463267645,
2.65338707632273E-15));
#119319=DIRECTION('ref_axis',(0.0914257765947348,-0.86985815903272,-0.484755722543072));
#119320=DIRECTION('',(0.104528463267644,-0.994521895368274,-1.47193748793052E-17));
#119321=DIRECTION('',(0.0522647556052278,-0.497265932938971,0.866022509672734));
#119322=DIRECTION('center_axis',(0.994521796395258,0.104529404915842,1.63998884832503E-6));
#119323=DIRECTION('ref_axis',(0.0905292105225956,-0.86132790107014,0.499918702270942));
#119324=DIRECTION('',(0.104528463267644,-0.994521895368274,-1.47193748793052E-17));
#119325=DIRECTION('center_axis',(0.994521994347068,0.104527521530174,1.64014401740936E-6));
#119326=DIRECTION('ref_axis',(0.0905261736006642,-0.861299008823645,-0.499969028333385));
#119327=DIRECTION('',(0.0522647719724824,-0.497266088663036,-0.866022419268942));
#119328=DIRECTION('',(0.104528463267644,-0.994521895368274,-1.47193748793052E-17));
#119329=DIRECTION('center_axis',(-0.994521895368274,-0.104528463267644,
1.40045497140052E-16));
#119330=DIRECTION('ref_axis',(1.55536281769216E-16,-1.40045497140052E-16,
1.));
#119331=DIRECTION('center_axis',(0.994521895368274,0.104528463267644,-4.41082526921583E-15));
#119332=DIRECTION('ref_axis',(0.0914257765929005,-0.86985815901529,-0.484755722574695));
#119333=DIRECTION('',(-0.0553921607193094,0.527021204990428,0.848045021223097));
#119334=DIRECTION('',(0.104528463267644,-0.994521895368274,-1.55536281769216E-16));
#119335=DIRECTION('',(-0.0553922155203033,0.527021726387038,-0.848044693619256));
#119336=DIRECTION('center_axis',(0.994521895368273,0.104528463267653,1.47142340632461E-14));
#119337=DIRECTION('ref_axis',(0.0914259726180641,-0.869860024070109,0.484752338886148));
#119338=DIRECTION('',(-0.104528463267644,0.994521895368274,1.47193748793052E-17));
#119339=DIRECTION('',(-0.0522647719724787,0.497266088663077,0.866022419268918));
#119340=DIRECTION('center_axis',(-0.99452179637225,-0.104529405134733,1.64037043048663E-6));
#119341=DIRECTION('ref_axis',(0.0905292212563007,-0.86132800319214,-0.499918524377491));
#119342=DIRECTION('',(-0.104528463267644,0.994521895368274,1.47193748793052E-17));
#119343=DIRECTION('center_axis',(-0.994521994324975,-0.104527521740383,
1.63977755580007E-6));
#119344=DIRECTION('ref_axis',(0.0905261624996592,-0.86129890320238,0.499969212297581));
#119345=DIRECTION('',(-0.0522647556052262,0.497265932938956,-0.866022509672743));
#119346=DIRECTION('',(-0.104528463267644,0.994521895368274,1.47193748793052E-17));
#119347=DIRECTION('center_axis',(-1.40816906889909E-16,1.4081690688991E-16,
-1.));
#119348=DIRECTION('ref_axis',(0.,1.,1.40816906889911E-16));
#119349=DIRECTION('',(1.04744440165294E-14,1.,1.40816906889909E-16));
#119350=DIRECTION('',(-1.04744440165294E-14,-1.,-1.40816906889909E-16));
#119351=DIRECTION('center_axis',(-1.,1.04744440165294E-14,1.4081690688991E-16));
#119352=DIRECTION('ref_axis',(1.40816906889909E-16,-1.40816906889911E-16,
1.));
#119353=DIRECTION('center_axis',(-1.,1.0218985244156E-14,-3.06110401690849E-16));
#119354=DIRECTION('ref_axis',(9.08643805832666E-15,0.874651456244175,-0.484752338921582));
#119355=DIRECTION('',(-5.41813057753239E-15,-0.529924709392051,0.84804469361924));
#119356=DIRECTION('',(1.04744440165294E-14,1.,1.40816906889909E-16));
#119357=DIRECTION('',(-5.67613898822991E-15,-0.529924185123396,-0.84804502122311));
#119358=DIRECTION('center_axis',(-1.,1.053745470252E-14,1.67445974214341E-16));
#119359=DIRECTION('ref_axis',(9.29775073408821E-15,0.874649580953058,0.484755722543468));
#119360=DIRECTION('',(-1.04744440165294E-14,-1.,1.4749788077992E-30));
#119361=DIRECTION('',(-5.23017107763447E-15,-0.500005012715,0.866022509672741));
#119362=DIRECTION('center_axis',(0.999999999998207,9.4683525304529E-7,1.63998886848176E-6));
#119363=DIRECTION('ref_axis',(1.66712501830529E-10,-0.866072335961381,0.499918702273076));
#119364=DIRECTION('',(-1.04744440165294E-14,-1.,1.4749788077992E-30));
#119365=DIRECTION('center_axis',(0.999999999998207,-9.46924657962836E-7,
1.64014403941177E-6));
#119366=DIRECTION('ref_axis',(-5.65192953370995E-11,-0.866043284547938,
-0.499969028330174));
#119367=DIRECTION('',(-5.36780659828042E-15,-0.50000516929684,-0.866022419268946));
#119368=DIRECTION('',(-1.04744440165294E-14,-1.,1.4749788077992E-30));
#119369=DIRECTION('center_axis',(-1.,1.04744440165294E-14,1.4081690688991E-16));
#119370=DIRECTION('ref_axis',(1.40816906889909E-16,-1.40816906889911E-16,
1.));
#119371=DIRECTION('center_axis',(1.,-1.03422010861309E-14,-3.74411322160043E-16));
#119372=DIRECTION('ref_axis',(9.22729987696341E-15,0.874649580936984,0.484755722572471));
#119373=DIRECTION('',(5.62453772470057E-15,0.529924185123411,0.8480450212231));
#119374=DIRECTION('',(-1.04744440165294E-14,-1.,-1.40816906889909E-16));
#119375=DIRECTION('',(5.41813057753243E-15,0.529924709392042,-0.848044693619246));
#119376=DIRECTION('center_axis',(1.,-1.04142386870038E-14,9.91450061389626E-17));
#119377=DIRECTION('ref_axis',(9.15688980706914E-15,0.874651456262602,-0.484752338888334));
#119378=DIRECTION('',(1.04744440165294E-14,1.,-1.4749788077992E-30));
#119379=DIRECTION('',(5.50544266490316E-15,0.500005169296855,0.866022419268938));
#119380=DIRECTION('center_axis',(-0.999999999998206,-9.4705534023739E-7,
1.64037042763668E-6));
#119381=DIRECTION('ref_axis',(1.66964445788292E-10,-0.86607243864958,-0.499918524373292));
#119382=DIRECTION('',(1.04744440165294E-14,1.,-1.4749788077992E-30));
#119383=DIRECTION('center_axis',(-0.999999999998207,9.46713293518364E-7,
1.6397775892974E-6));
#119384=DIRECTION('ref_axis',(-5.6280035541352E-11,-0.866043178343455,0.499969212296884));
#119385=DIRECTION('',(5.09253499664393E-15,0.500005012714985,-0.86602250967275));
#119386=DIRECTION('',(1.04744440165294E-14,1.,-1.4749788077992E-30));
#119387=DIRECTION('center_axis',(-1.26097532010602E-16,1.40045497140051E-16,
-1.));
#119388=DIRECTION('ref_axis',(0.,1.,1.40045497140051E-16));
#119389=DIRECTION('',(0.104528463267664,0.994521895368272,1.26097532010602E-16));
#119390=DIRECTION('center_axis',(1.26097532010602E-16,-1.40045497140051E-16,
1.));
#119391=DIRECTION('ref_axis',(1.94422256072357E-12,1.,1.40045497139806E-16));
#119392=DIRECTION('',(-0.104528463267664,-0.994521895368272,-1.26097532010602E-16));
#119393=DIRECTION('center_axis',(-1.26097532010602E-16,1.40045497140051E-16,
-1.));
#119394=DIRECTION('ref_axis',(2.83644037037302E-33,1.,1.40045497140051E-16));
#119395=DIRECTION('center_axis',(-0.994521895368272,0.104528463267664,1.40045497140051E-16));
#119396=DIRECTION('ref_axis',(1.26097532010602E-16,-1.40045497140051E-16,
1.));
#119397=DIRECTION('center_axis',(-0.994521895368272,0.104528463267663,-3.37703732557294E-15));
#119398=DIRECTION('ref_axis',(0.0914259726159238,0.869860024049577,-0.484752338923395));
#119399=DIRECTION('',(-0.0553922155203143,-0.527021726387072,0.848044693619234));
#119400=DIRECTION('',(0.104528463267664,0.994521895368272,1.26097532010602E-16));
#119401=DIRECTION('',(-0.0553921607193168,-0.527021204990409,-0.848045021223109));
#119402=DIRECTION('center_axis',(-0.994521895368273,0.104528463267661,6.06488474588053E-15));
#119403=DIRECTION('ref_axis',(0.0914257765946926,0.869858159032147,0.484755722544108));
#119404=DIRECTION('',(-0.104528463267664,-0.994521895368272,1.4719374879308E-17));
#119405=DIRECTION('',(-0.0522647556052199,-0.497265932938945,0.86602250967275));
#119406=DIRECTION('center_axis',(0.994521994337725,-0.104527521619066,1.63998887836188E-6));
#119407=DIRECTION('ref_axis',(0.0905292101911294,0.86132790110626,-0.499918702268733));
#119408=DIRECTION('',(-0.104528463267664,-0.994521895368272,1.4719374879308E-17));
#119409=DIRECTION('center_axis',(0.994521796385908,-0.104529405004792,1.64014407563316E-6));
#119410=DIRECTION('ref_axis',(0.0905261737131063,0.861299008812056,0.49996902833299));
#119411=DIRECTION('',(-0.052264771972493,-0.497266088662982,-0.866022419268971));
#119412=DIRECTION('',(-0.104528463267664,-0.994521895368272,1.4719374879308E-17));
#119413=DIRECTION('center_axis',(-0.994521895368272,0.104528463267664,1.40045497140051E-16));
#119414=DIRECTION('ref_axis',(1.26097532010602E-16,-1.40045497140051E-16,
1.));
#119415=DIRECTION('center_axis',(0.994521895368272,-0.104528463267665,2.27433177943941E-15));
#119416=DIRECTION('ref_axis',(0.0914257765929865,0.869858159015916,0.484755722573557));
#119417=DIRECTION('',(0.055392160719317,0.527021204990424,0.848045021223099));
#119418=DIRECTION('',(-0.104528463267664,-0.994521895368272,-1.26097532010602E-16));
#119419=DIRECTION('',(0.055392215520313,0.527021726387063,-0.84804469361924));
#119420=DIRECTION('center_axis',(0.994521895368273,-0.104528463267659,1.52655870960609E-14));
#119421=DIRECTION('ref_axis',(0.0914259726179232,0.869860024068582,-0.484752338888914));
#119422=DIRECTION('',(0.104528463267664,0.994521895368272,-1.4719374879308E-17));
#119423=DIRECTION('',(0.0522647719724912,0.497266088663035,0.866022419268941));
#119424=DIRECTION('center_axis',(-0.994521994360727,0.104527521400209,1.64037038848631E-6));
#119425=DIRECTION('ref_axis',(0.0905292209241732,0.861328003226788,0.499918524377938));
#119426=DIRECTION('',(0.104528463267664,0.994521895368272,-1.4719374879308E-17));
#119427=DIRECTION('center_axis',(-0.994521796408004,0.104529404794571,1.63977760137252E-6));
#119428=DIRECTION('ref_axis',(0.0905261626116839,0.861298903191368,-0.499969212296267));
#119429=DIRECTION('',(0.0522647556052202,0.497265932938941,-0.866022509672752));
#119430=DIRECTION('',(0.104528463267664,0.994521895368272,-1.4719374879308E-17));
#119431=DIRECTION('center_axis',(-1.11539425682701E-16,1.37739719617121E-16,
-1.));
#119432=DIRECTION('ref_axis',(0.,1.,1.37739719617121E-16));
#119433=DIRECTION('',(0.20791169081777,0.978147600733803,1.11539425682701E-16));
#119434=DIRECTION('center_axis',(1.11539425682701E-16,-1.37739719617121E-16,
1.));
#119435=DIRECTION('ref_axis',(2.43272069155864E-12,1.,1.3773971961685E-16));
#119436=DIRECTION('',(-0.20791169081777,-0.978147600733803,-1.11539425682701E-16));
#119437=DIRECTION('center_axis',(-1.11539425682701E-16,1.37739719617121E-16,
-1.));
#119438=DIRECTION('ref_axis',(2.25178493903968E-33,1.,1.37739719617121E-16));
#119439=DIRECTION('center_axis',(-0.978147600733803,0.20791169081777,1.37739719617121E-16));
#119440=DIRECTION('ref_axis',(1.11539425682701E-16,-1.37739719617121E-16,
1.));
#119441=DIRECTION('center_axis',(-0.978147600733801,0.207911690817781,1.02000311058135E-14));
#119442=DIRECTION('ref_axis',(0.181850263143849,0.855538223403061,-0.484752338922513));
#119443=DIRECTION('',(-0.110177542335815,-0.518344583061384,0.848044693619245));
#119444=DIRECTION('',(0.20791169081777,0.978147600733803,1.11539425682701E-16));
#119445=DIRECTION('',(-0.110177433334236,-0.518344070249262,-0.848045021223112));
#119446=DIRECTION('center_axis',(-0.978147600733804,0.207911690817767,8.33921652558567E-15));
#119447=DIRECTION('ref_axis',(0.181849873248782,0.855536389091008,0.484755722545409));
#119448=DIRECTION('',(-0.20791169081777,-0.978147600733803,2.92774812072098E-17));
#119449=DIRECTION('',(-0.103956887610934,-0.489078703542056,0.866022509672739));
#119450=DIRECTION('center_axis',(0.978147797590165,-0.20791076467278,1.63998884165523E-6));
#119451=DIRECTION('ref_axis',(0.180066563577549,0.847146577519057,-0.4999187022698));
#119452=DIRECTION('',(-0.20791169081777,-0.978147600733803,2.92774812072098E-17));
#119453=DIRECTION('center_axis',(0.978147403855348,-0.207912617049456,1.64014400359551E-6));
#119454=DIRECTION('ref_axis',(0.180060523666452,0.847118160897777,0.499969028334887));
#119455=DIRECTION('',(-0.103956920166134,-0.489078856702197,-0.866022419268949));
#119456=DIRECTION('',(-0.20791169081777,-0.978147600733803,2.92774812072098E-17));
#119457=DIRECTION('center_axis',(-0.978147600733803,0.20791169081777,1.37739719617121E-16));
#119458=DIRECTION('ref_axis',(1.11539425682701E-16,-1.37739719617121E-16,
1.));
#119459=DIRECTION('center_axis',(0.9781476007338,-0.207911690817786,3.72163382090106E-14));
#119460=DIRECTION('ref_axis',(0.181849873245445,0.855536389075333,0.484755722574325));
#119461=DIRECTION('',(0.110177433334237,0.518344070249278,0.848045021223102));
#119462=DIRECTION('',(-0.20791169081777,-0.978147600733803,-1.11539425682701E-16));
#119463=DIRECTION('',(0.110177542335821,0.518344583061396,-0.848044693619237));
#119464=DIRECTION('center_axis',(0.9781476007338,-0.207911690817784,-3.30122628397866E-14));
#119465=DIRECTION('ref_axis',(0.181850263147825,0.855538223421808,-0.484752338887935));
#119466=DIRECTION('',(0.20791169081777,0.978147600733803,-2.92774812072098E-17));
#119467=DIRECTION('',(0.103956920166143,0.489078856702196,0.866022419268949));
#119468=DIRECTION('center_axis',(-0.978147797635926,0.207910764457488,1.64037041047626E-6));
#119469=DIRECTION('ref_axis',(0.180066584926733,0.847146677960321,0.499918524375339));
#119470=DIRECTION('',(0.20791169081777,0.978147600733803,-2.92774812072098E-17));
#119471=DIRECTION('center_axis',(-0.978147403899287,0.207912616842742,1.63977762800927E-6));
#119472=DIRECTION('ref_axis',(0.180060501585904,0.847118057018156,-0.499969212294534));
#119473=DIRECTION('',(0.103956887610928,0.489078703542026,-0.866022509672757));
#119474=DIRECTION('',(0.20791169081777,0.978147600733803,-2.92774812072098E-17));
#119475=DIRECTION('center_axis',(-9.73020895656121E-17,1.33924836902177E-16,
-1.));
#119476=DIRECTION('ref_axis',(0.,1.,1.33924836902177E-16));
#119477=DIRECTION('',(0.309016994374957,0.95105651629515,9.73020895656121E-17));
#119478=DIRECTION('center_axis',(9.73020895656121E-17,-1.33924836902177E-16,
1.));
#119479=DIRECTION('ref_axis',(2.04991579266789E-12,1.,1.33924836901977E-16));
#119480=DIRECTION('',(-0.309016994374957,-0.95105651629515,-9.73020895656121E-17));
#119481=DIRECTION('center_axis',(-9.73020895656121E-17,1.33924836902177E-16,
-1.));
#119482=DIRECTION('ref_axis',(1.59316208980364E-33,1.,1.33924836902177E-16));
#119483=DIRECTION('center_axis',(-0.95105651629515,0.309016994374957,1.33924836902177E-16));
#119484=DIRECTION('ref_axis',(9.73020895656121E-17,-1.33924836902177E-16,
1.));
#119485=DIRECTION('center_axis',(-0.951056516295151,0.309016994374954,-1.10270606549325E-15));
#119486=DIRECTION('ref_axis',(0.270282164133958,0.831842966947162,-0.484752338923296));
#119487=DIRECTION('',(-0.163755740941356,-0.503988348013123,0.84804469361924));
#119488=DIRECTION('',(0.309016994374957,0.95105651629515,9.73020895656121E-17));
#119489=DIRECTION('',(-0.163755578933431,-0.503987849404003,-0.84804502122311));
#119490=DIRECTION('center_axis',(-0.951056516295154,0.309016994374946,1.48865352853434E-14));
#119491=DIRECTION('ref_axis',(0.270281584636996,0.831841183438903,0.484755722545985));
#119492=DIRECTION('',(-0.309016994374957,-0.95105651629515,4.35148173242984E-17));
#119493=DIRECTION('',(-0.15451004620158,-0.475533025522863,0.866022509672732));
#119494=DIRECTION('center_axis',(0.95105680888162,-0.309016093880593,1.6399887814086E-6));
#119495=DIRECTION('ref_axis',(0.26763107001171,0.823683738751163,-0.499918702271972));
#119496=DIRECTION('',(-0.309016994374957,-0.95105651629515,4.35148173242984E-17));
#119497=DIRECTION('center_axis',(0.951056223677639,-0.30901789495325,1.64014400927579E-6));
#119498=DIRECTION('ref_axis',(0.267622092842645,0.823656109143276,0.499969028334239));
#119499=DIRECTION('',(-0.154510094588055,-0.475533174441005,-0.866022419268954));
#119500=DIRECTION('',(-0.309016994374957,-0.95105651629515,4.35148173242984E-17));
#119501=DIRECTION('center_axis',(-0.95105651629515,0.309016994374957,1.33924836902177E-16));
#119502=DIRECTION('ref_axis',(9.73020895656121E-17,-1.33924836902177E-16,
1.));
#119503=DIRECTION('center_axis',(0.951056516295148,-0.309016994374965,3.72163382090098E-15));
#119504=DIRECTION('ref_axis',(0.270281584632176,0.831841183424041,0.484755722574176));
#119505=DIRECTION('',(0.163755578933424,0.503987849404003,0.848045021223111));
#119506=DIRECTION('',(-0.309016994374957,-0.95105651629515,-9.73020895656121E-17));
#119507=DIRECTION('',(0.163755740941359,0.503988348013123,-0.84804469361924));
#119508=DIRECTION('center_axis',(0.951056516295157,-0.309016994374937,1.83324883410909E-14));
#119509=DIRECTION('ref_axis',(0.27028216414016,0.83184296696627,-0.48475233888705));
#119510=DIRECTION('',(0.309016994374957,0.95105651629515,-4.35148173242984E-17));
#119511=DIRECTION('',(0.15451009458807,0.475533174440996,0.866022419268956));
#119512=DIRECTION('center_axis',(-0.951056808949647,0.309016093671226,1.64037042347201E-6));
#119513=DIRECTION('ref_axis',(0.267631101743148,0.823683836411319,0.499918524376203));
#119514=DIRECTION('',(0.309016994374957,0.95105651629515,-4.35148173242984E-17));
#119515=DIRECTION('center_axis',(-0.951056223742963,0.309017894752208,1.63977752868973E-6));
#119516=DIRECTION('ref_axis',(0.26762206002332,0.82365600813657,-0.499969212301523));
#119517=DIRECTION('',(0.154510046201593,0.475533025522812,-0.866022509672758));
#119518=DIRECTION('',(0.309016994374957,0.95105651629515,-4.35148173242984E-17));
#119519=DIRECTION('center_axis',(-8.35415108931894E-17,1.28642645648558E-16,
-1.));
#119520=DIRECTION('ref_axis',(0.,1.,1.28642645648558E-16));
#119521=DIRECTION('',(0.40673664307581,0.913545457642596,8.35415108931894E-17));
#119522=DIRECTION('center_axis',(8.35415108931894E-17,-1.28642645648558E-16,
1.));
#119523=DIRECTION('ref_axis',(2.68585154117318E-12,1.,1.28642645648334E-16));
#119524=DIRECTION('',(-0.40673664307581,-0.913545457642596,-8.35415108931894E-17));
#119525=DIRECTION('center_axis',(-8.35415108931894E-17,1.28642645648558E-16,
-1.));
#119526=DIRECTION('ref_axis',(9.26572950507599E-34,1.,1.28642645648558E-16));
#119527=DIRECTION('center_axis',(-0.913545457642596,0.40673664307581,1.28642645648558E-16));
#119528=DIRECTION('ref_axis',(8.35415108931894E-17,-1.28642645648558E-16,
1.));
#119529=DIRECTION('center_axis',(-0.913545457642591,0.406736643075822,2.2329797826238E-14));
#119530=DIRECTION('ref_axis',(0.355752797174115,0.799033864872324,-0.484752338921629));
#119531=DIRECTION('',(-0.215539797381059,-0.484110311157677,0.848044693619239));
#119532=DIRECTION('',(0.40673664307581,0.913545457642596,8.35415108931894E-17));
#119533=DIRECTION('',(-0.215539584141775,-0.484109832214432,-0.84804502122311));
#119534=DIRECTION('center_axis',(-0.913545457642595,0.406736643075814,-9.64868027753666E-16));
#119535=DIRECTION('ref_axis',(0.355752034424621,0.799032151708906,0.484755722542993));
#119536=DIRECTION('',(-0.40673664307581,-0.913545457642596,5.72753959967212E-17));
#119537=DIRECTION('',(-0.20337036039277,-0.456777308164325,0.866022509672739));
#119538=DIRECTION('center_axis',(0.913545842753538,-0.406735778098066,1.6399887859702E-6));
#119539=DIRECTION('ref_axis',(0.352263354438556,0.79119644857774,-0.499918702268347));
#119540=DIRECTION('',(-0.40673664307581,-0.913545457642596,5.72753959967212E-17));
#119541=DIRECTION('center_axis',(0.913545072491979,-0.406737508133851,1.64014419087578E-6));
#119542=DIRECTION('ref_axis',(0.352251538365721,0.791169908694829,0.499969028335555));
#119543=DIRECTION('',(-0.203370424080349,-0.456777451208949,-0.866022419268945));
#119544=DIRECTION('',(-0.40673664307581,-0.913545457642596,5.72753959967212E-17));
#119545=DIRECTION('center_axis',(-0.913545457642596,0.40673664307581,1.28642645648558E-16));
#119546=DIRECTION('ref_axis',(8.35415108931894E-17,-1.28642645648558E-16,
1.));
#119547=DIRECTION('center_axis',(0.913545457642598,-0.406736643075806,-1.40595055456267E-14));
#119548=DIRECTION('ref_axis',(0.355752034417943,0.799032151693909,0.484755722572614));
#119549=DIRECTION('',(0.215539584141768,0.484109832214442,0.848045021223106));
#119550=DIRECTION('',(-0.40673664307581,-0.913545457642596,-8.35415108931894E-17));
#119551=DIRECTION('',(0.215539797381042,0.484110311157656,-0.848044693619255));
#119552=DIRECTION('center_axis',(0.9135454576426,-0.406736643075802,2.04000622141478E-14));
#119553=DIRECTION('ref_axis',(0.355752797181682,0.799033864889318,-0.484752338888064));
#119554=DIRECTION('',(0.40673664307581,0.913545457642596,-5.72753959967212E-17));
#119555=DIRECTION('',(0.20337042408034,0.456777451208963,0.866022419268939));
#119556=DIRECTION('center_axis',(-0.91354584284308,0.406735777896949,1.64037046486978E-6));
#119557=DIRECTION('ref_axis',(0.352263396203314,0.791196542383525,0.499918524377384));
#119558=DIRECTION('',(0.40673664307581,0.913545457642596,-5.72753959967212E-17));
#119559=DIRECTION('center_axis',(-0.913545072577964,0.406737507940728,1.6397775875592E-6));
#119560=DIRECTION('ref_axis',(0.352251495168338,0.791169811672393,-0.499969212302058));
#119561=DIRECTION('',(0.203370360392774,0.456777308164295,-0.866022509672753));
#119562=DIRECTION('',(0.40673664307581,0.913545457642596,-5.72753959967212E-17));
#119563=DIRECTION('center_axis',(-7.04084534449538E-17,1.2195101864901E-16,
-1.));
#119564=DIRECTION('ref_axis',(0.,1.,1.2195101864901E-16));
#119565=DIRECTION('',(0.50000000000001,0.866025403784433,7.04084534449538E-17));
#119566=DIRECTION('center_axis',(7.04084534449538E-17,-1.2195101864901E-16,
1.));
#119567=DIRECTION('ref_axis',(2.63700172808967E-12,1.,1.21951018648824E-16));
#119568=DIRECTION('',(-0.50000000000001,-0.866025403784433,-7.04084534449538E-17));
#119569=DIRECTION('center_axis',(-7.04084534449538E-17,1.2195101864901E-16,
-1.));
#119570=DIRECTION('ref_axis',(3.09764893063008E-34,1.,1.2195101864901E-16));
#119571=DIRECTION('center_axis',(-0.866025403784433,0.50000000000001,1.2195101864901E-16));
#119572=DIRECTION('ref_axis',(7.04084534449538E-17,-1.2195101864901E-16,
1.));
#119573=DIRECTION('center_axis',(-0.866025403784415,0.500000000000041,4.54866252015975E-14));
#119574=DIRECTION('ref_axis',(0.437325728121414,0.757470380563304,-0.484752338924073));
#119575=DIRECTION('',(-0.264962354696027,-0.458928260426592,0.848044693619245));
#119576=DIRECTION('',(0.50000000000001,0.866025403784433,7.04084534449538E-17));
#119577=DIRECTION('',(-0.264962092561705,-0.458927806396623,-0.848045021223111));
#119578=DIRECTION('center_axis',(-0.866025403784399,0.500000000000068,-9.57976113269888E-14));
#119579=DIRECTION('ref_axis',(0.437324790477049,0.757468756515617,0.484755722541663));
#119580=DIRECTION('',(-0.50000000000001,-0.866025403784433,7.04084534449566E-17));
#119581=DIRECTION('',(-0.250002506357495,-0.433017043030775,0.866022509672731));
#119582=DIRECTION('center_axis',(0.866025877200486,-0.499999180015767,1.63998881574967E-6));
#119583=DIRECTION('ref_axis',(0.433036167836511,0.750040644541146,-0.499918702272451));
#119584=DIRECTION('',(-0.50000000000001,-0.866025403784433,7.04084534449566E-17));
#119585=DIRECTION('center_axis',(0.866024930320552,-0.50000082005992,1.6401440734818E-6));
#119586=DIRECTION('ref_axis',(0.433021642322727,0.750015485166862,0.499969028330801));
#119587=DIRECTION('',(-0.250002584648428,-0.433017178634614,-0.866022419268938));
#119588=DIRECTION('',(-0.50000000000001,-0.866025403784433,7.04084534449566E-17));
#119589=DIRECTION('center_axis',(-0.866025403784433,0.50000000000001,1.2195101864901E-16));
#119590=DIRECTION('ref_axis',(7.04084534449538E-17,-1.2195101864901E-16,
1.));
#119591=DIRECTION('center_axis',(0.866025403784456,-0.49999999999997,-7.02975277281265E-14));
#119592=DIRECTION('ref_axis',(0.437324790468275,0.757468756500457,0.484755722573268));
#119593=DIRECTION('',(0.264962092561697,0.458927806396632,0.848045021223108));
#119594=DIRECTION('',(-0.50000000000001,-0.866025403784433,-7.04084534449538E-17));
#119595=DIRECTION('',(0.264962354696035,0.458928260426609,-0.848044693619234));
#119596=DIRECTION('center_axis',(0.866025403784424,-0.500000000000025,-2.88081959645749E-14));
#119597=DIRECTION('ref_axis',(0.43732572813103,0.757470380579976,-0.484752338889345));
#119598=DIRECTION('',(0.50000000000001,0.866025403784433,-7.04084534449566E-17));
#119599=DIRECTION('',(0.250002584648412,0.433017178634587,0.866022419268956));
#119600=DIRECTION('center_axis',(-0.866025877310554,0.499999179825123,1.64037042562383E-6));
#119601=DIRECTION('ref_axis',(0.433036219179545,0.75004073347043,0.499918524375547));
#119602=DIRECTION('',(0.50000000000001,0.866025403784433,-7.04084534449566E-17));
#119603=DIRECTION('center_axis',(-0.86602493042628,0.500000819876797,1.63977742833608E-6));
#119604=DIRECTION('ref_axis',(0.433021589220767,0.750015393192006,-0.499969212295879));
#119605=DIRECTION('',(0.250002506357492,0.43301704303074,-0.866022509672749));
#119606=DIRECTION('',(0.50000000000001,0.866025403784433,-7.04084534449566E-17));
#119607=DIRECTION('center_axis',(-5.80468057465775E-17,1.13923270769251E-16,
-1.));
#119608=DIRECTION('ref_axis',(0.,1.,1.13923270769251E-16));
#119609=DIRECTION('',(0.587785252292482,0.809016994374941,5.80468057465775E-17));
#119610=DIRECTION('center_axis',(5.80468057465775E-17,-1.13923270769251E-16,
1.));
#119611=DIRECTION('ref_axis',(2.03917556295366E-34,1.,1.13923270769251E-16));
#119612=DIRECTION('',(-0.587785252292482,-0.809016994374941,-5.80468057465775E-17));
#119613=DIRECTION('center_axis',(-5.80468057465775E-17,1.13923270769251E-16,
-1.));
#119614=DIRECTION('ref_axis',(-2.10605807273598E-34,1.,1.13923270769251E-16));
#119615=DIRECTION('center_axis',(-0.809016994374941,0.587785252292482,1.13923270769251E-16));
#119616=DIRECTION('ref_axis',(5.80468057465775E-17,-1.13923270769251E-16,
1.));
#119617=DIRECTION('center_axis',(-0.809016994374934,0.587785252292492,1.68162674987722E-14));
#119618=DIRECTION('ref_axis',(0.514107226875554,0.707607892255063,-0.484752338924398));
#119619=DIRECTION('',(-0.311481929006024,-0.428718095637375,0.848044693619239));
#119620=DIRECTION('',(0.587785252292482,0.809016994374941,5.80468057465775E-17));
#119621=DIRECTION('',(-0.31148162084864,-0.428717671495099,-0.848045021223122));
#119622=DIRECTION('center_axis',(-0.809016994374973,0.587785252292438,7.37434849783257E-14));
#119623=DIRECTION('ref_axis',(0.514106124608232,0.707606375114275,0.484755722542748));
#119624=DIRECTION('',(-0.587785252292482,-0.809016994374941,8.2770101143333E-17));
#119625=DIRECTION('',(-0.293895572546169,-0.404512552559093,0.866022509672749));
#119626=DIRECTION('center_axis',(0.809017550909317,-0.587784486285578,1.63998898495591E-6));
#119627=DIRECTION('ref_axis',(0.509064546362255,0.700667238249452,-0.499918702271557));
#119628=DIRECTION('',(-0.587785252292482,-0.809016994374941,8.2770101143333E-17));
#119629=DIRECTION('center_axis',(0.809016437785117,-0.587786018369602,1.64014408828489E-6));
#119630=DIRECTION('ref_axis',(0.509047470548778,0.700643735028728,0.49996902833364));
#119631=DIRECTION('',(-0.293895664582707,-0.404512679236446,-0.866022419268948));
#119632=DIRECTION('',(-0.587785252292482,-0.809016994374941,8.2770101143333E-17));
#119633=DIRECTION('center_axis',(-0.809016994374941,0.587785252292482,1.13923270769251E-16));
#119634=DIRECTION('ref_axis',(5.80468057465775E-17,-1.13923270769251E-16,
1.));
#119635=DIRECTION('center_axis',(0.809016994374913,-0.58778525229252,1.10546308309721E-13));
#119636=DIRECTION('ref_axis',(0.514106124598513,0.707606375100899,0.48475572257258));
#119637=DIRECTION('',(0.311481620848643,0.42871767149512,0.84804502122311));
#119638=DIRECTION('',(-0.587785252292482,-0.809016994374941,-5.80468057465775E-17));
#119639=DIRECTION('',(0.31148192900604,0.428718095637378,-0.848044693619232));
#119640=DIRECTION('center_axis',(0.809016994374959,-0.587785252292457,6.781642303623E-14));
#119641=DIRECTION('ref_axis',(0.514107226887019,0.707607892270838,-0.484752338889211));
#119642=DIRECTION('',(0.587785252292482,0.809016994374941,-8.2770101143333E-17));
#119643=DIRECTION('',(0.293895664582671,0.404512679236479,0.866022419268945));
#119644=DIRECTION('center_axis',(-0.809017551038645,0.587784486107572,1.64037042958252E-6));
#119645=DIRECTION('ref_axis',(0.509064606719795,0.700667321324917,0.499918524374308));
#119646=DIRECTION('',(0.587785252292482,0.809016994374941,-8.2770101143333E-17));
#119647=DIRECTION('center_axis',(-0.809016437909404,0.587786018198536,1.63977756741941E-6));
#119648=DIRECTION('ref_axis',(0.509047408125916,0.700643649111502,-0.499969212292123));
#119649=DIRECTION('',(0.293895572546207,0.404512552559083,-0.866022509672741));
#119650=DIRECTION('',(0.587785252292482,0.809016994374941,-8.2770101143333E-17));
#119651=DIRECTION('center_axis',(-4.65920045970846E-17,1.04647355694968E-16,
-1.));
#119652=DIRECTION('ref_axis',(0.,1.,1.04647355694968E-16));
#119653=DIRECTION('',(0.669130606358867,0.743144825477386,4.65920045970846E-17));
#119654=DIRECTION('center_axis',(4.65920045970846E-17,-1.04647355694968E-16,
1.));
#119655=DIRECTION('ref_axis',(-5.08215691752411E-12,1.,1.04647355695205E-16));
#119656=DIRECTION('',(-0.669130606358867,-0.743144825477386,-4.65920045970846E-17));
#119657=DIRECTION('center_axis',(-4.65920045970846E-17,1.04647355694968E-16,
-1.));
#119658=DIRECTION('ref_axis',(-6.01228899222973E-34,1.,1.04647355694968E-16));
#119659=DIRECTION('center_axis',(-0.743144825477386,0.669130606358867,1.04647355694968E-16));
#119660=DIRECTION('ref_axis',(4.65920045970846E-17,-1.04647355694968E-16,
1.));
#119661=DIRECTION('center_axis',(-0.743144825477412,0.669130606358838,-6.09245101184987E-14));
#119662=DIRECTION('ref_axis',(0.585256059268807,0.649992703803544,-0.484752338922985));
#119663=DIRECTION('',(-0.354588842120043,-0.393810805677315,0.84804469361924));
#119664=DIRECTION('',(0.669130606358867,0.743144825477386,4.65920045970846E-17));
#119665=DIRECTION('',(-0.354588491315847,-0.393810416069776,-0.848045021223108));
#119666=DIRECTION('center_axis',(-0.743144825477402,0.66913060635885,4.3281222959236E-14));
#119667=DIRECTION('ref_axis',(0.585254804454853,0.649991310191455,0.484755722542919));
#119668=DIRECTION('',(-0.669130606358867,-0.743144825477386,9.42249022928259E-17));
#119669=DIRECTION('',(-0.334568657340454,-0.371576137911918,0.866022509672739));
#119670=DIRECTION('center_axis',(0.743145459032515,-0.669129902721933,1.6399889188559E-6));
#119671=DIRECTION('ref_axis',(0.579515507189717,0.643617175071609,-0.499918702270166));
#119672=DIRECTION('',(-0.669130606358867,-0.743144825477386,9.42249022928259E-17));
#119673=DIRECTION('center_axis',(0.743144191859766,-0.669131310059846,1.6401440772679E-6));
#119674=DIRECTION('ref_axis',(0.579496068163272,0.643595585511955,0.499969028333588));
#119675=DIRECTION('',(-0.334568762114156,-0.371576254274936,-0.86602241926893));
#119676=DIRECTION('',(-0.669130606358867,-0.743144825477386,9.42249022928259E-17));
#119677=DIRECTION('center_axis',(-0.743144825477386,0.669130606358867,1.04647355694968E-16));
#119678=DIRECTION('ref_axis',(4.65920045970846E-17,-1.04647355694968E-16,
1.));
#119679=DIRECTION('center_axis',(0.743144825477406,-0.669130606358846,-1.31222051759166E-13));
#119680=DIRECTION('ref_axis',(0.585254804443108,0.649991310178355,0.484755722574664));
#119681=DIRECTION('',(0.354588491315847,0.39381041606979,0.848045021223102));
#119682=DIRECTION('',(-0.669130606358867,-0.743144825477386,-4.65920045970846E-17));
#119683=DIRECTION('',(0.354588842120062,0.393810805677307,-0.848044693619236));
#119684=DIRECTION('center_axis',(0.743144825477372,-0.669130606358882,-7.33299533643765E-14));
#119685=DIRECTION('ref_axis',(0.585256059281577,0.649992703817746,-0.484752338888524));
#119686=DIRECTION('',(0.669130606358867,0.743144825477386,-9.42249022928259E-17));
#119687=DIRECTION('',(0.334568762114183,0.371576254274923,0.866022419268924));
#119688=DIRECTION('center_axis',(-0.743145459179742,0.66912990255842,1.64037033353259E-6));
#119689=DIRECTION('ref_axis',(0.579515575898918,0.643617251381315,0.499918524376628));
#119690=DIRECTION('',(0.669130606358867,0.743144825477386,-9.42249022928259E-17));
#119691=DIRECTION('center_axis',(-0.7431441920012,0.669131309902768,1.63977763833729E-6));
#119692=DIRECTION('ref_axis',(0.579495997100135,0.643595506588717,-0.499969212295851));
#119693=DIRECTION('',(0.33456865734047,0.371576137911861,-0.866022509672757));
#119694=DIRECTION('',(0.669130606358867,0.743144825477386,-9.42249022928259E-17));
#119695=DIRECTION('center_axis',(-3.61695511949404E-17,9.42249022928235E-17,
-1.));
#119696=DIRECTION('ref_axis',(0.,1.,9.42249022928235E-17));
#119697=DIRECTION('',(0.743144825477402,0.66913060635885,3.61695511949404E-17));
#119698=DIRECTION('center_axis',(3.61695511949404E-17,-9.42249022928235E-17,
1.));
#119699=DIRECTION('ref_axis',(1.24700250125898E-12,1.,9.42249022927784E-17));
#119700=DIRECTION('',(-0.743144825477402,-0.66913060635885,-3.61695511949404E-17));
#119701=DIRECTION('center_axis',(-3.61695511949404E-17,9.42249022928235E-17,
-1.));
#119702=DIRECTION('ref_axis',(-8.43711753644599E-34,1.,9.42249022928235E-17));
#119703=DIRECTION('center_axis',(-0.66913060635885,0.743144825477402,9.42249022928235E-17));
#119704=DIRECTION('ref_axis',(3.61695511949404E-17,-9.42249022928235E-17,
1.));
#119705=DIRECTION('center_axis',(-0.669130606358838,0.743144825477412,6.09245101184987E-14));
#119706=DIRECTION('ref_axis',(0.649992703804063,0.585256059269274,-0.484752338921726));
#119707=DIRECTION('',(-0.393810805677328,-0.35458884212003,0.84804469361924));
#119708=DIRECTION('',(0.743144825477402,0.66913060635885,3.61695511949404E-17));
#119709=DIRECTION('',(-0.393810416069783,-0.354588491315852,-0.848045021223102));
#119710=DIRECTION('center_axis',(-0.669130606358808,0.74314482547744,-6.53353493078877E-14));
#119711=DIRECTION('ref_axis',(0.649991310191615,0.585254804454945,0.484755722542594));
#119712=DIRECTION('',(-0.743144825477402,-0.66913060635885,1.0464735569497E-16));
#119713=DIRECTION('',(-0.371576137911934,-0.334568657340433,0.86602250967274));
#119714=DIRECTION('center_axis',(0.669131309993433,-0.743144191919564,1.63998895207813E-6));
#119715=DIRECTION('ref_axis',(0.643617174847078,0.579515507436224,-0.499918702273481));
#119716=DIRECTION('',(-0.743144825477402,-0.66913060635885,1.0464735569497E-16));
#119717=DIRECTION('center_axis',(0.669129902655543,-0.743145459092292,1.64014393853014E-6));
#119718=DIRECTION('ref_axis',(0.643595585587858,0.579496068079491,0.499969028332989));
#119719=DIRECTION('',(-0.371576254274944,-0.334568762114131,-0.866022419268936));
#119720=DIRECTION('',(-0.743144825477402,-0.66913060635885,1.0464735569497E-16));
#119721=DIRECTION('center_axis',(-0.66913060635885,0.743144825477402,9.42249022928235E-17));
#119722=DIRECTION('ref_axis',(3.61695511949404E-17,-9.42249022928235E-17,
1.));
#119723=DIRECTION('center_axis',(0.669130606358856,-0.743144825477396,-2.31568326633862E-14));
#119724=DIRECTION('ref_axis',(0.649991310178348,0.585254804443017,0.484755722574783));
#119725=DIRECTION('',(0.393810416069767,0.354588491315837,0.848045021223116));
#119726=DIRECTION('',(-0.743144825477402,-0.66913060635885,-3.61695511949404E-17));
#119727=DIRECTION('',(0.393810805677295,0.354588842120035,-0.848044693619253));
#119728=DIRECTION('center_axis',(0.669130606358837,-0.743144825477414,2.34325038946298E-14));
#119729=DIRECTION('ref_axis',(0.649992703818525,0.585256059282238,-0.484752338886682));
#119730=DIRECTION('',(0.743144825477402,0.66913060635885,-1.0464735569497E-16));
#119731=DIRECTION('',(0.371576254274883,0.33456876211414,0.866022419268959));
#119732=DIRECTION('center_axis',(-0.66913131015695,0.743144191772332,1.64037043491853E-6));
#119733=DIRECTION('ref_axis',(0.643617251158306,0.579515576147492,0.499918524375589));
#119734=DIRECTION('',(0.743144825477402,0.66913060635885,-1.0464735569497E-16));
#119735=DIRECTION('center_axis',(-0.669129902812644,0.743145458950839,1.6397773398599E-6));
#119736=DIRECTION('ref_axis',(0.643595506659834,0.579495997012642,-0.499969212305713));
#119737=DIRECTION('',(0.371576137911907,0.334568657340444,-0.866022509672747));
#119738=DIRECTION('',(0.743144825477402,0.66913060635885,-1.0464735569497E-16));
#119739=DIRECTION('center_axis',(-2.68936361206573E-17,8.27701011433304E-17,
-1.));
#119740=DIRECTION('ref_axis',(0.,1.,8.27701011433304E-17));
#119741=DIRECTION('',(0.809016994374955,0.587785252292463,2.68936361206573E-17));
#119742=DIRECTION('center_axis',(2.68936361206573E-17,-8.27701011433304E-17,
1.));
#119743=DIRECTION('ref_axis',(-7.43345068374092E-34,1.,8.27701011433304E-17));
#119744=DIRECTION('',(-0.809016994374955,-0.587785252292463,-2.68936361206573E-17));
#119745=DIRECTION('center_axis',(-2.68936361206573E-17,8.27701011433304E-17,
-1.));
#119746=DIRECTION('ref_axis',(-9.35397677642637E-34,1.,8.27701011433303E-17));
#119747=DIRECTION('center_axis',(-0.587785252292463,0.809016994374955,8.27701011433303E-17));
#119748=DIRECTION('ref_axis',(2.68936361206573E-17,-8.27701011433304E-17,
1.));
#119749=DIRECTION('center_axis',(-0.587785252292444,0.809016994374969,1.57135614332808E-14));
#119750=DIRECTION('ref_axis',(0.707607892255383,0.514107226875742,-0.484752338923732));
#119751=DIRECTION('',(-0.428718095637369,-0.31148192900601,0.848044693619247));
#119752=DIRECTION('',(0.809016994374955,0.587785252292463,2.68936361206573E-17));
#119753=DIRECTION('',(-0.428717671495124,-0.311481620848633,-0.848045021223112));
#119754=DIRECTION('center_axis',(-0.587785252292501,0.809016994374927,9.01462414501431E-14));
#119755=DIRECTION('ref_axis',(0.707606375113487,0.514106124607646,0.484755722544519));
#119756=DIRECTION('',(-0.809016994374955,-0.587785252292463,1.13923270769253E-16));
#119757=DIRECTION('',(-0.404512552559104,-0.293895572546205,0.866022509672732));
#119758=DIRECTION('center_axis',(0.587786018297244,-0.809016437837688,1.63998890629073E-6));
#119759=DIRECTION('ref_axis',(0.700667238054952,0.509064546633043,-0.499918702268419));
#119760=DIRECTION('',(-0.809016994374955,-0.587785252292463,1.13923270769253E-16));
#119761=DIRECTION('center_axis',(0.58778448621328,-0.809017550961845,1.64014403044851E-6));
#119762=DIRECTION('ref_axis',(0.700643735097504,0.509047470458993,0.499969028328675));
#119763=DIRECTION('',(-0.40451267923645,-0.293895664582675,-0.866022419268957));
#119764=DIRECTION('',(-0.809016994374955,-0.587785252292463,1.13923270769253E-16));
#119765=DIRECTION('center_axis',(-0.587785252292463,0.809016994374955,8.27701011433303E-17));
#119766=DIRECTION('ref_axis',(2.68936361206573E-17,-8.27701011433304E-17,
1.));
#119767=DIRECTION('center_axis',(0.587785252292418,-0.809016994374988,4.46596058508136E-14));
#119768=DIRECTION('ref_axis',(0.707606375100562,0.514106124598224,0.484755722573379));
#119769=DIRECTION('',(0.428717671495113,0.311481620848634,0.848045021223117));
#119770=DIRECTION('',(-0.809016994374955,-0.587785252292463,-2.68936361206573E-17));
#119771=DIRECTION('',(0.428718095637379,0.311481929006014,-0.84804469361924));
#119772=DIRECTION('center_axis',(0.587785252292438,-0.809016994374973,-5.15515085681819E-14));
#119773=DIRECTION('ref_axis',(0.707607892271254,0.514107226887285,-0.484752338888322));
#119774=DIRECTION('',(0.809016994374955,0.587785252292463,-1.13923270769253E-16));
#119775=DIRECTION('',(0.404512679236446,0.293895664582707,0.866022419268948));
#119776=DIRECTION('center_axis',(-0.587786018475273,0.809016437708342,1.64037041133668E-6));
#119777=DIRECTION('ref_axis',(0.700667321128982,0.509064606990169,0.499918524373603));
#119778=DIRECTION('',(0.809016994374955,0.587785252292463,-1.13923270769253E-16));
#119779=DIRECTION('center_axis',(-0.587784486384226,0.809017550837646,1.63977767104282E-6));
#119780=DIRECTION('ref_axis',(0.700643649177376,0.50904740803465,-0.499969212292732));
#119781=DIRECTION('',(0.404512552559085,0.293895572546138,-0.866022509672763));
#119782=DIRECTION('',(0.809016994374955,0.587785252292463,-1.13923270769253E-16));
#119783=DIRECTION('center_axis',(-1.88658882408992E-17,7.04084534449537E-17,
-1.));
#119784=DIRECTION('ref_axis',(0.,1.,7.04084534449537E-17));
#119785=DIRECTION('',(0.866025403784445,0.499999999999989,1.88658882408992E-17));
#119786=DIRECTION('center_axis',(1.88658882408992E-17,-7.04084534449537E-17,
1.));
#119787=DIRECTION('ref_axis',(2.39808173319034E-12,1.,7.04084534449084E-17));
#119788=DIRECTION('',(-0.866025403784445,-0.499999999999989,-1.88658882408992E-17));
#119789=DIRECTION('center_axis',(-1.88658882408992E-17,7.04084534449537E-17,
-1.));
#119790=DIRECTION('ref_axis',(-8.89395021849233E-34,1.,7.04084534449537E-17));
#119791=DIRECTION('center_axis',(-0.499999999999989,0.866025403784445,7.04084534449537E-17));
#119792=DIRECTION('ref_axis',(1.88658882408992E-17,-7.04084534449537E-17,
1.));
#119793=DIRECTION('center_axis',(-0.500000000000001,0.866025403784438,3.58379471285317E-15));
#119794=DIRECTION('ref_axis',(0.757470380565452,0.437325728122635,-0.484752338919614));
#119795=DIRECTION('',(-0.458928260426618,-0.264962354696007,0.848044693619237));
#119796=DIRECTION('',(0.866025403784445,0.499999999999989,1.88658882408991E-17));
#119797=DIRECTION('',(-0.458927806396625,-0.264962092561694,-0.848045021223113));
#119798=DIRECTION('center_axis',(-0.49999999999998,0.86602540378445,-3.36325426817012E-14));
#119799=DIRECTION('ref_axis',(0.757468756515611,0.437324790477015,0.484755722541703));
#119800=DIRECTION('',(-0.866025403784445,-0.499999999999989,1.21951018649011E-16));
#119801=DIRECTION('',(-0.433017043030788,-0.2500025063575,0.866022509672722));
#119802=DIRECTION('center_axis',(0.50000081998251,-0.866024930365246,1.63998892746333E-6));
#119803=DIRECTION('ref_axis',(0.750040644373928,0.433036168124944,-0.499918702273488));
#119804=DIRECTION('',(-0.866025403784445,-0.499999999999989,1.21951018649011E-16));
#119805=DIRECTION('center_axis',(0.499999179938316,-0.866025877245202,1.64014398672678E-6));
#119806=DIRECTION('ref_axis',(0.750015485223452,0.43302164222488,0.499969028330653));
#119807=DIRECTION('',(-0.433017178634633,-0.250002584648383,-0.866022419268941));
#119808=DIRECTION('',(-0.866025403784445,-0.499999999999989,1.21951018649011E-16));
#119809=DIRECTION('center_axis',(-0.499999999999989,0.866025403784445,7.04084534449537E-17));
#119810=DIRECTION('ref_axis',(1.88658882408992E-17,-7.04084534449537E-17,
1.));
#119811=DIRECTION('center_axis',(0.499999999999953,-0.866025403784466,8.87678585429635E-14));
#119812=DIRECTION('ref_axis',(0.757468756498903,0.437324790467367,0.484755722576515));
#119813=DIRECTION('',(0.458927806396636,0.264962092561686,0.848045021223109));
#119814=DIRECTION('',(-0.866025403784445,-0.499999999999989,-1.88658882408991E-17));
#119815=DIRECTION('',(0.458928260426592,0.264962354696007,-0.848044693619251));
#119816=DIRECTION('center_axis',(0.499999999999964,-0.866025403784459,-4.21785070103366E-14));
#119817=DIRECTION('ref_axis',(0.757470380579776,0.437325728130884,-0.48475233888979));
#119818=DIRECTION('',(0.866025403784445,0.499999999999989,-1.21951018649011E-16));
#119819=DIRECTION('',(0.433017178634602,0.250002584648404,0.866022419268951));
#119820=DIRECTION('center_axis',(-0.500000820173088,0.866024930255214,1.64037045316471E-6));
#119821=DIRECTION('ref_axis',(0.750040733303908,0.433036219468976,0.499918524374674));
#119822=DIRECTION('',(0.866025403784445,0.499999999999989,-1.21951018649011E-16));
#119823=DIRECTION('center_axis',(-0.499999180121355,0.866025877139526,1.63977753161604E-6));
#119824=DIRECTION('ref_axis',(0.750015393246846,0.433021589122425,-0.499969212298786));
#119825=DIRECTION('',(0.43301704303074,0.250002506357492,-0.866022509672749));
#119826=DIRECTION('',(0.866025403784445,0.499999999999989,-1.21951018649011E-16));
#119827=DIRECTION('center_axis',(-1.2174261241351E-17,5.72753959967181E-17,
-1.));
#119828=DIRECTION('ref_axis',(0.,1.,5.72753959967181E-17));
#119829=DIRECTION('',(0.913545457642606,0.406736643075789,1.2174261241351E-17));
#119830=DIRECTION('center_axis',(1.2174261241351E-17,-5.72753959967181E-17,
1.));
#119831=DIRECTION('ref_axis',(-7.04858393874019E-12,1.,5.72753959968039E-17));
#119832=DIRECTION('',(-0.913545457642606,-0.406736643075789,-1.2174261241351E-17));
#119833=DIRECTION('center_axis',(-1.2174261241351E-17,5.72753959967181E-17,
-1.));
#119834=DIRECTION('ref_axis',(6.97285633565874E-34,1.,5.72753959967181E-17));
#119835=DIRECTION('center_axis',(-0.406736643075789,0.913545457642606,5.72753959967181E-17));
#119836=DIRECTION('ref_axis',(1.2174261241351E-17,-5.72753959967181E-17,
1.));
#119837=DIRECTION('center_axis',(-0.406736643075804,0.913545457642599,-8.27029549119977E-16));
#119838=DIRECTION('ref_axis',(0.79903386487198,0.355752797173954,-0.484752338922314));
#119839=DIRECTION('',(-0.484110311157678,-0.215539797381027,0.848044693619247));
#119840=DIRECTION('',(0.913545457642606,0.406736643075789,1.2174261241351E-17));
#119841=DIRECTION('',(-0.484109832214435,-0.215539584141758,-0.848045021223113));
#119842=DIRECTION('center_axis',(-0.406736643075777,0.913545457642611,-2.15027731899433E-14));
#119843=DIRECTION('ref_axis',(0.799032151708161,0.355752034424262,0.484755722544485));
#119844=DIRECTION('',(-0.913545457642606,-0.406736643075789,1.2864264564856E-16));
#119845=DIRECTION('',(-0.456777308164333,-0.203370360392756,0.866022509672737));
#119846=DIRECTION('center_axis',(0.40673750805212,-0.913545072528368,1.63998882745409E-6));
#119847=DIRECTION('ref_axis',(0.791196448443063,0.352263354743605,-0.499918702266544));
#119848=DIRECTION('',(-0.913545457642606,-0.406736643075789,1.2864264564856E-16));
#119849=DIRECTION('center_axis',(0.40673577801635,-0.913545842789919,1.64014404421889E-6));
#119850=DIRECTION('ref_axis',(0.7911699087431,0.352251538263499,0.49996902833119));
#119851=DIRECTION('',(-0.456777451208922,-0.203370424080335,-0.866022419268962));
#119852=DIRECTION('',(-0.913545457642606,-0.406736643075789,1.2864264564856E-16));
#119853=DIRECTION('center_axis',(-0.406736643075789,0.913545457642606,5.72753959967181E-17));
#119854=DIRECTION('ref_axis',(1.2174261241351E-17,-5.72753959967181E-17,
1.));
#119855=DIRECTION('center_axis',(0.406736643075782,-0.913545457642609,-4.4108252692162E-15));
#119856=DIRECTION('ref_axis',(0.799032151693547,0.355752034417747,0.484755722573354));
#119857=DIRECTION('',(0.48410983221443,0.215539584141761,0.848045021223115));
#119858=DIRECTION('',(-0.913545457642606,-0.406736643075789,-1.2174261241351E-17));
#119859=DIRECTION('',(0.484110311157677,0.215539797381033,-0.848044693619246));
#119860=DIRECTION('center_axis',(0.406736643075817,-0.913545457642593,4.39704043669829E-14));
#119861=DIRECTION('ref_axis',(0.799033864889481,0.355752797181736,-0.484752338887755));
#119862=DIRECTION('',(0.913545457642606,0.406736643075789,-1.2864264564856E-16));
#119863=DIRECTION('',(0.45677745120894,0.203370424080363,0.866022419268946));
#119864=DIRECTION('center_axis',(-0.406737508253128,0.913545072438873,1.64037036124584E-6));
#119865=DIRECTION('ref_axis',(0.791196542247866,0.35226339650843,0.499918524377089));
#119866=DIRECTION('',(0.913545457642606,0.406736643075789,-1.2864264564856E-16));
#119867=DIRECTION('center_axis',(-0.406735778209486,0.913545842703931,1.63977751199266E-6));
#119868=DIRECTION('ref_axis',(0.79116981172108,0.352251495066775,-0.499969212296569));
#119869=DIRECTION('',(0.456777308164311,0.203370360392764,-0.866022509672747));
#119870=DIRECTION('',(0.913545457642606,0.406736643075789,-1.2864264564856E-16));
#119871=DIRECTION('center_axis',(-6.89206998773264E-18,4.35148173242952E-17,
-1.));
#119872=DIRECTION('ref_axis',(0.,1.,4.35148173242952E-17));
#119873=DIRECTION('',(0.951056516295158,0.309016994374935,6.89206998773264E-18));
#119874=DIRECTION('center_axis',(6.89206998773264E-18,-4.35148173242952E-17,
1.));
#119875=DIRECTION('ref_axis',(-6.90292267790937E-12,1.,4.35148173243428E-17));
#119876=DIRECTION('',(-0.951056516295158,-0.309016994374935,-6.89206998773264E-18));
#119877=DIRECTION('center_axis',(-6.89206998773264E-18,4.35148173242952E-17,
-1.));
#119878=DIRECTION('ref_axis',(2.99907166502443E-34,1.,4.35148173242952E-17));
#119879=DIRECTION('center_axis',(-0.309016994374935,0.951056516295158,4.35148173242952E-17));
#119880=DIRECTION('ref_axis',(6.89206998773264E-18,-4.35148173242952E-17,
1.));
#119881=DIRECTION('center_axis',(-0.309016994374926,0.95105651629516,4.13514774560007E-15));
#119882=DIRECTION('ref_axis',(0.831842966945941,0.270282164133536,-0.484752338925627));
#119883=DIRECTION('',(-0.503988348013125,-0.163755740941349,0.84804469361924));
#119884=DIRECTION('',(0.951056516295158,0.309016994374935,6.89206998773264E-18));
#119885=DIRECTION('',(-0.503987849404011,-0.163755578933422,-0.848045021223107));
#119886=DIRECTION('center_axis',(-0.309016994374912,0.951056516295165,-4.49352824353855E-14));
#119887=DIRECTION('ref_axis',(0.831841183439609,0.270281584637207,0.484755722544655));
#119888=DIRECTION('',(-0.951056516295158,-0.309016994374935,1.33924836902178E-16));
#119889=DIRECTION('',(-0.475533025522885,-0.154510046201587,0.866022509672719));
#119890=DIRECTION('center_axis',(0.30901789486823,-0.951056223705265,1.63998885189632E-6));
#119891=DIRECTION('ref_axis',(0.8236837386523,0.26763107033019,-0.499918702264364));
#119892=DIRECTION('',(-0.951056516295158,-0.309016994374935,1.33924836902178E-16));
#119893=DIRECTION('center_axis',(0.309016093795513,-0.951056808909264,1.64014401908765E-6));
#119894=DIRECTION('ref_axis',(0.823656109180483,0.267622092735848,0.499969028330108));
#119895=DIRECTION('',(-0.475533174441007,-0.154510094588029,-0.866022419268957));
#119896=DIRECTION('',(-0.951056516295158,-0.309016994374935,1.33924836902178E-16));
#119897=DIRECTION('center_axis',(-0.309016994374935,0.951056516295158,4.35148173242952E-17));
#119898=DIRECTION('ref_axis',(6.89206998773264E-18,-4.35148173242952E-17,
1.));
#119899=DIRECTION('center_axis',(0.309016994374914,-0.951056516295165,2.96352322775422E-14));
#119900=DIRECTION('ref_axis',(0.831841183423017,0.27028158463181,0.484755722576136));
#119901=DIRECTION('',(0.503987849404013,0.163755578933423,0.848045021223105));
#119902=DIRECTION('',(-0.951056516295158,-0.309016994374935,-6.89206998773264E-18));
#119903=DIRECTION('',(0.503988348013112,0.163755740941343,-0.848044693619249));
#119904=DIRECTION('center_axis',(0.309016994374935,-0.951056516295158,1.92973561485194E-14));
#119905=DIRECTION('ref_axis',(0.831842966965813,0.27028216413999,-0.484752338887928));
#119906=DIRECTION('',(0.951056516295158,0.309016994374935,-1.33924836902178E-16));
#119907=DIRECTION('',(0.475533174441017,0.154510094588048,0.866022419268948));
#119908=DIRECTION('center_axis',(-0.309017895077531,0.951056223637258,1.64037041727555E-6));
#119909=DIRECTION('ref_axis',(0.823683836307394,0.267631102060501,0.49991852437754));
#119910=DIRECTION('',(0.951056516295158,0.309016994374935,-1.33924836902178E-16));
#119911=DIRECTION('center_axis',(-0.309016093996569,0.951056808843938,1.63977753815644E-6));
#119912=DIRECTION('ref_axis',(0.823656008171523,0.267622059916318,-0.499969212301216));
#119913=DIRECTION('',(0.47553302552284,0.15451004620159,-0.866022509672743));
#119914=DIRECTION('',(0.951056516295158,0.309016994374935,-1.33924836902178E-16));
#119915=DIRECTION('center_axis',(-3.07718727278846E-18,2.92774812072065E-17,
-1.));
#119916=DIRECTION('ref_axis',(0.,1.,2.92774812072065E-17));
#119917=DIRECTION('',(0.978147600733808,0.207911690817747,3.07718727278847E-18));
#119918=DIRECTION('center_axis',(3.07718727278846E-18,-2.92774812072065E-17,
1.));
#119919=DIRECTION('ref_axis',(2.25419682919892E-12,1.,2.92774812071996E-17));
#119920=DIRECTION('',(-0.978147600733808,-0.207911690817747,-3.07718727278847E-18));
#119921=DIRECTION('center_axis',(-3.07718727278846E-18,2.92774812072065E-17,
-1.));
#119922=DIRECTION('ref_axis',(9.00922925501191E-35,1.,2.92774812072065E-17));
#119923=DIRECTION('center_axis',(-0.207911690817747,0.978147600733808,2.92774812072065E-17));
#119924=DIRECTION('ref_axis',(3.07718727278847E-18,-2.92774812072065E-17,
1.));
#119925=DIRECTION('center_axis',(-0.207911690817745,0.978147600733809,2.75676516373318E-15));
#119926=DIRECTION('ref_axis',(0.855538223402063,0.18185026314361,-0.484752338924365));
#119927=DIRECTION('',(-0.518344583061394,-0.110177542335804,0.84804469361924));
#119928=DIRECTION('',(0.978147600733808,0.207911690817747,3.07718727278847E-18));
#119929=DIRECTION('',(-0.51834407024927,-0.110177433334225,-0.848045021223109));
#119930=DIRECTION('center_axis',(-0.207911690817745,0.978147600733809,7.0986719184735E-15));
#119931=DIRECTION('ref_axis',(0.855536389092103,0.181849873248987,0.484755722543399));
#119932=DIRECTION('',(-0.978147600733808,-0.207911690817747,1.37739719617122E-16));
#119933=DIRECTION('',(-0.489078703542048,-0.103956887610933,0.866022509672743));
#119934=DIRECTION('center_axis',(0.20791261696197,-0.978147403873944,1.63998878691659E-6));
#119935=DIRECTION('ref_axis',(0.847146577451719,0.1800665639041,-0.499918702266288));
#119936=DIRECTION('',(-0.978147600733808,-0.207911690817747,1.37739719617122E-16));
#119937=DIRECTION('center_axis',(0.207910764585278,-0.978147797608764,1.64014406418637E-6));
#119938=DIRECTION('ref_axis',(0.847118160921327,0.180060523555876,0.499969028334809));
#119939=DIRECTION('',(-0.489078856702224,-0.103956920166124,-0.866022419268935));
#119940=DIRECTION('',(-0.978147600733808,-0.207911690817747,1.37739719617122E-16));
#119941=DIRECTION('center_axis',(-0.207911690817747,0.978147600733808,2.92774812072065E-17));
#119942=DIRECTION('ref_axis',(3.07718727278847E-18,-2.92774812072065E-17,
1.));
#119943=DIRECTION('center_axis',(0.20791169081776,-0.978147600733805,-3.47352489950765E-14));
#119944=DIRECTION('ref_axis',(0.85553638907458,0.181849873245263,0.484755722575723));
#119945=DIRECTION('',(0.51834407024926,0.110177433334222,0.848045021223115));
#119946=DIRECTION('',(-0.978147600733808,-0.207911690817747,-3.07718727278847E-18));
#119947=DIRECTION('',(0.518344583061389,0.110177542335803,-0.848044693619244));
#119948=DIRECTION('center_axis',(0.207911690817756,-0.978147600733806,2.61203499296049E-14));
#119949=DIRECTION('ref_axis',(0.85553822342184,0.18185026314781,-0.484752338887884));
#119950=DIRECTION('',(0.978147600733808,0.207911690817747,-1.37739719617122E-16));
#119951=DIRECTION('',(0.48907885670221,0.103956920166112,0.866022419268945));
#119952=DIRECTION('center_axis',(-0.207912617177295,0.978147403828174,1.64037044739867E-6));
#119953=DIRECTION('ref_axis',(0.847146677890568,0.180066585253285,0.499918524375919));
#119954=DIRECTION('',(0.978147600733808,0.207911690817747,-1.37739719617122E-16));
#119955=DIRECTION('center_axis',(-0.207910764792043,0.978147797564815,1.63977759590673E-6));
#119956=DIRECTION('ref_axis',(0.847118057037499,0.180060501474941,-0.499969212301723));
#119957=DIRECTION('',(0.489078703542054,0.103956887610909,-0.866022509672743));
#119958=DIRECTION('',(0.978147600733808,0.207911690817747,-1.37739719617122E-16));
#119959=DIRECTION('center_axis',(-7.71409749858844E-19,1.47193748793047E-17,
-1.));
#119960=DIRECTION('ref_axis',(0.,1.,1.47193748793047E-17));
#119961=DIRECTION('',(0.994521895368275,0.10452846326764,7.71409749858844E-19));
#119962=DIRECTION('center_axis',(7.71409749858844E-19,-1.47193748793047E-17,
1.));
#119963=DIRECTION('ref_axis',(2.20623519453511E-12,1.,1.4719374879303E-17));
#119964=DIRECTION('',(-0.994521895368275,-0.10452846326764,-7.71409749858844E-19));
#119965=DIRECTION('center_axis',(-7.71409749858844E-19,1.47193748793047E-17,
-1.));
#119966=DIRECTION('ref_axis',(1.1354669293723E-35,1.,1.47193748793047E-17));
#119967=DIRECTION('center_axis',(-0.10452846326764,0.994521895368275,1.47193748793047E-17));
#119968=DIRECTION('ref_axis',(7.71409749858844E-19,-1.47193748793047E-17,
1.));
#119969=DIRECTION('center_axis',(-0.104528463267633,0.994521895368276,1.65405909823986E-14));
#119970=DIRECTION('ref_axis',(0.869860024050798,0.0914259726160318,-0.484752338921184));
#119971=DIRECTION('',(-0.527021726387079,-0.0553922155203004,0.848044693619231));
#119972=DIRECTION('',(0.994521895368275,0.10452846326764,7.71409749858844E-19));
#119973=DIRECTION('',(-0.527021204990416,-0.0553921607193045,-0.848045021223105));
#119974=DIRECTION('center_axis',(-0.104528463267648,0.994521895368274,1.14061184709465E-14));
#119975=DIRECTION('ref_axis',(0.869858159032786,0.0914257765947394,0.484755722542953));
#119976=DIRECTION('',(-0.994521895368275,-0.10452846326764,1.40045497140052E-16));
#119977=DIRECTION('',(-0.497265932938979,-0.0522647556052154,0.86602250967273));
#119978=DIRECTION('center_axis',(0.104529404915859,-0.994521796395256,1.63998887728709E-6));
#119979=DIRECTION('ref_axis',(0.861327901070781,0.0905292105226631,-0.499918702269825));
#119980=DIRECTION('',(-0.994521895368275,-0.10452846326764,1.40045497140052E-16));
#119981=DIRECTION('center_axis',(0.104527521530148,-0.99452199434707,1.64014406315375E-6));
#119982=DIRECTION('ref_axis',(0.861299008823921,0.0905261736006938,0.499969028332904));
#119983=DIRECTION('',(-0.497266088662994,-0.0522647719724685,-0.866022419268966));
#119984=DIRECTION('',(-0.994521895368275,-0.10452846326764,1.40045497140052E-16));
#119985=DIRECTION('center_axis',(-0.10452846326764,0.994521895368275,1.47193748793047E-17));
#119986=DIRECTION('ref_axis',(7.71409749858844E-19,-1.47193748793047E-17,
1.));
#119987=DIRECTION('center_axis',(0.104528463267637,-0.994521895368275,3.58379553123799E-15));
#119988=DIRECTION('ref_axis',(0.869858159015688,0.0914257765929404,0.484755722573974));
#119989=DIRECTION('',(0.527021204990409,0.0553921607193052,0.848045021223109));
#119990=DIRECTION('',(-0.994521895368275,-0.10452846326764,-7.71409749858844E-19));
#119991=DIRECTION('',(0.52702172638707,0.0553922155203008,-0.848044693619237));
#119992=DIRECTION('center_axis',(0.104528463267642,-0.994521895368275,3.99730948790747E-15));
#119993=DIRECTION('ref_axis',(0.86986002406859,0.0914259726178999,-0.484752338888904));
#119994=DIRECTION('',(0.994521895368275,0.10452846326764,-1.40045497140052E-16));
#119995=DIRECTION('',(0.497266088663062,0.0522647719724771,0.866022419268927));
#119996=DIRECTION('center_axis',(-0.104529405134726,0.994521796372251,1.6403704192978E-6));
#119997=DIRECTION('ref_axis',(0.861328003192725,0.0905292212563617,0.499918524376472));
#119998=DIRECTION('',(0.994521895368275,0.10452846326764,-1.40045497140052E-16));
#119999=DIRECTION('center_axis',(-0.104527521740357,0.994521994324977,1.6397776076981E-6));
#120000=DIRECTION('ref_axis',(0.861298903199663,0.0905261624993766,-0.499969212302312));
#120001=DIRECTION('',(0.497265932938956,0.0522647556052086,-0.866022509672744));
#120002=DIRECTION('',(0.994521895368275,0.10452846326764,-1.40045497140052E-16));
#120003=DIRECTION('center_axis',(0.994521895368273,-0.104528463267654,7.71409749859047E-19));
#120004=DIRECTION('ref_axis',(0.104528463267654,0.994521895368273,1.12125269189207E-32));
#120005=DIRECTION('center_axis',(-0.994521895368273,0.104528463267654,-7.71409749859047E-19));
#120006=DIRECTION('ref_axis',(-0.104528463267654,-0.994521895368273,-5.60397807285558E-36));
#120007=DIRECTION('center_axis',(0.978147600733806,-0.20791169081776,3.07718727278885E-18));
#120008=DIRECTION('ref_axis',(0.20791169081776,0.978147600733805,5.3337836051253E-32));
#120009=DIRECTION('center_axis',(-0.978147600733806,0.20791169081776,-3.07718727278885E-18));
#120010=DIRECTION('ref_axis',(-0.20791169081776,-0.978147600733805,2.17629115865656E-35));
#120011=DIRECTION('center_axis',(0.951056516295153,-0.309016994374948,6.89206998773323E-18));
#120012=DIRECTION('ref_axis',(0.309016994374948,0.951056516295153,2.1129734794752E-32));
#120013=DIRECTION('center_axis',(-0.951056516295153,0.309016994374948,-6.89206998773323E-18));
#120014=DIRECTION('ref_axis',(-0.309016994374948,-0.951056516295153,-3.51157074825093E-34));
#120015=DIRECTION('center_axis',(0.913545457642601,-0.406736643075801,1.21742612413517E-17));
#120016=DIRECTION('ref_axis',(0.406736643075801,0.913545457642601,-1.81348366517715E-31));
#120017=DIRECTION('center_axis',(-0.913545457642601,0.406736643075801,-1.21742612413517E-17));
#120018=DIRECTION('ref_axis',(-0.406736643075801,-0.9135454576426,1.31266757742093E-34));
#120019=DIRECTION('center_axis',(0.866025403784438,-0.500000000000001,1.88658882409001E-17));
#120020=DIRECTION('ref_axis',(0.500000000000001,0.866025403784438,8.56587576076706E-32));
#120021=DIRECTION('center_axis',(-0.866025403784438,0.500000000000001,-1.88658882409001E-17));
#120022=DIRECTION('ref_axis',(-0.500000000000001,-0.866025403784438,6.22903900877646E-34));
#120023=DIRECTION('center_axis',(0.809016994374947,-0.587785252292474,2.68936361206584E-17));
#120024=DIRECTION('ref_axis',(0.587785252292474,0.809016994374947,-4.93427012362456E-31));
#120025=DIRECTION('center_axis',(-0.809016994374947,0.587785252292474,-2.68936361206584E-17));
#120026=DIRECTION('ref_axis',(-0.587785252292474,-0.809016994374947,1.15372963471371E-33));
#120027=DIRECTION('center_axis',(0.743144825477393,-0.669130606358859,3.61695511949416E-17));
#120028=DIRECTION('ref_axis',(0.669130606358859,0.743144825477393,6.27086406135521E-31));
#120029=DIRECTION('center_axis',(-0.743144825477393,0.669130606358859,-3.61695511949416E-17));
#120030=DIRECTION('ref_axis',(-0.669130606358859,-0.743144825477393,7.72831234962683E-33));
#120031=DIRECTION('center_axis',(0.669130606358857,-0.743144825477395,4.6592004597086E-17));
#120032=DIRECTION('ref_axis',(0.743144825477396,0.669130606358857,-6.54359212772961E-31));
#120033=DIRECTION('center_axis',(-0.669130606358857,0.743144825477395,-4.6592004597086E-17));
#120034=DIRECTION('ref_axis',(-0.743144825477395,-0.669130606358857,4.37914107422688E-33));
#120035=DIRECTION('center_axis',(0.587785252292471,-0.809016994374949,5.8046805746579E-17));
#120036=DIRECTION('ref_axis',(0.809016994374949,0.587785252292471,1.26008547401877E-30));
#120037=DIRECTION('center_axis',(-0.587785252292471,0.809016994374949,-5.8046805746579E-17));
#120038=DIRECTION('ref_axis',(-0.809016994374949,-0.587785252292472,3.97684690788254E-33));
#120039=DIRECTION('center_axis',(0.499999999999998,-0.86602540378444,7.04084534449555E-17));
#120040=DIRECTION('ref_axis',(0.86602540378444,0.499999999999998,-7.7693955971012E-31));
#120041=DIRECTION('center_axis',(-0.499999999999998,0.86602540378444,-7.04084534449555E-17));
#120042=DIRECTION('ref_axis',(-0.86602540378444,-0.499999999999998,4.12230412422948E-33));
#120043=DIRECTION('center_axis',(0.406736643075798,-0.913545457642602,8.35415108931911E-17));
#120044=DIRECTION('ref_axis',(0.913545457642602,0.406736643075798,1.52177632324919E-30));
#120045=DIRECTION('center_axis',(-0.406736643075798,0.913545457642602,-8.35415108931911E-17));
#120046=DIRECTION('ref_axis',(-0.913545457642602,-0.406736643075798,-8.4716126159886E-33));
#120047=DIRECTION('center_axis',(0.309016994374945,-0.951056516295155,9.73020895656139E-17));
#120048=DIRECTION('ref_axis',(0.951056516295154,0.309016994374945,2.18819993268723E-32));
#120049=DIRECTION('center_axis',(-0.309016994374945,0.951056516295155,-9.73020895656139E-17));
#120050=DIRECTION('ref_axis',(-0.951056516295154,-0.309016994374945,-3.99634687419351E-33));
#120051=DIRECTION('center_axis',(0.207911690817756,-0.978147600733806,1.11539425682703E-16));
#120052=DIRECTION('ref_axis',(0.978147600733806,0.207911690817756,-1.55106258718425E-30));
#120053=DIRECTION('center_axis',(-0.207911690817756,0.978147600733806,-1.11539425682703E-16));
#120054=DIRECTION('ref_axis',(-0.978147600733806,-0.207911690817756,-8.73440025092029E-33));
#120055=DIRECTION('center_axis',(0.10452846326765,-0.994521895368274,1.26097532010604E-16));
#120056=DIRECTION('ref_axis',(0.994521895368274,0.10452846326765,-1.41047068150179E-30));
#120057=DIRECTION('center_axis',(-0.10452846326765,0.994521895368274,-1.26097532010604E-16));
#120058=DIRECTION('ref_axis',(-0.994521895368274,-0.10452846326765,6.75407294460559E-34));
#120059=DIRECTION('center_axis',(-3.49148133884313E-15,-1.,1.40816906889911E-16));
#120060=DIRECTION('ref_axis',(1.,-3.49148133884313E-15,4.91659602599735E-31));
#120061=DIRECTION('center_axis',(3.49148133884313E-15,1.,-1.40816906889911E-16));
#120062=DIRECTION('ref_axis',(-1.,3.49148133884313E-15,8.75811540203011E-47));
#120063=DIRECTION('center_axis',(-0.104528463267657,-0.994521895368273,
1.55536281769218E-16));
#120064=DIRECTION('ref_axis',(0.994521895368273,-0.104528463267657,2.79416186164968E-30));
#120065=DIRECTION('center_axis',(0.104528463267657,0.994521895368273,-1.55536281769218E-16));
#120066=DIRECTION('ref_axis',(-0.994521895368273,0.104528463267657,-2.13589730221744E-33));
#120067=DIRECTION('center_axis',(-0.207911690817763,-0.978147600733805,
1.70094388097119E-16));
#120068=DIRECTION('ref_axis',(0.978147600733805,-0.207911690817763,-3.06962581902968E-30));
#120069=DIRECTION('center_axis',(0.207911690817763,0.978147600733805,-1.70094388097119E-16));
#120070=DIRECTION('ref_axis',(-0.978147600733805,0.207911690817763,-1.74175573100342E-33));
#120071=DIRECTION('center_axis',(-0.309016994374951,-0.951056516295152,
1.84331724214208E-16));
#120072=DIRECTION('ref_axis',(0.951056516295152,-0.309016994374951,1.20064847815822E-30));
#120073=DIRECTION('center_axis',(0.309016994374951,0.951056516295152,-1.84331724214208E-16));
#120074=DIRECTION('ref_axis',(-0.951056516295152,0.309016994374951,-1.12286633426729E-32));
#120075=DIRECTION('center_axis',(-0.406736643075804,-0.913545457642599,
1.98092302886631E-16));
#120076=DIRECTION('ref_axis',(0.913545457642599,-0.406736643075804,-2.28374368880912E-30));
#120077=DIRECTION('center_axis',(0.406736643075804,0.913545457642599,-1.98092302886631E-16));
#120078=DIRECTION('ref_axis',(-0.913545457642599,0.406736643075804,-2.42004257715226E-33));
#120079=DIRECTION('center_axis',(-0.500000000000004,-0.866025403784436,
2.11225360334866E-16));
#120080=DIRECTION('ref_axis',(0.866025403784436,-0.500000000000004,1.67705471180066E-30));
#120081=DIRECTION('center_axis',(0.500000000000004,0.866025403784436,-2.11225360334866E-16));
#120082=DIRECTION('ref_axis',(-0.866025403784436,0.500000000000004,-2.24248448190466E-35));
#120083=DIRECTION('center_axis',(-0.587785252292477,-0.809016994374945,
2.23587008033243E-16));
#120084=DIRECTION('ref_axis',(0.809016994374945,-0.587785252292477,-3.32537644322472E-30));
#120085=DIRECTION('center_axis',(0.587785252292477,0.809016994374945,-2.23587008033243E-16));
#120086=DIRECTION('ref_axis',(-0.809016994374945,0.587785252292477,5.18779161054862E-33));
#120087=DIRECTION('center_axis',(-0.669130606358862,-0.743144825477391,
2.35041809182736E-16));
#120088=DIRECTION('ref_axis',(0.743144825477391,-0.669130606358862,4.90467981149431E-30));
#120089=DIRECTION('center_axis',(0.669130606358862,0.743144825477391,-2.35041809182736E-16));
#120090=DIRECTION('ref_axis',(-0.743144825477391,0.669130606358862,7.02183635389561E-33));
#120091=DIRECTION('center_axis',(-0.743144825477398,-0.669130606358854,
2.4546426258488E-16));
#120092=DIRECTION('ref_axis',(0.669130606358854,-0.743144825477398,-2.63996916307136E-30));
#120093=DIRECTION('center_axis',(0.743144825477398,0.669130606358854,-2.4546426258488E-16));
#120094=DIRECTION('ref_axis',(-0.669130606358854,0.743144825477398,-2.15782657736967E-33));
#120095=DIRECTION('center_axis',(-0.809016994374951,-0.587785252292469,
2.54740177659163E-16));
#120096=DIRECTION('ref_axis',(0.587785252292469,-0.80901699437495,6.34109604668436E-30));
#120097=DIRECTION('center_axis',(0.809016994374951,0.587785252292469,-2.54740177659163E-16));
#120098=DIRECTION('ref_axis',(-0.587785252292469,0.809016994374951,-1.15824900225317E-32));
#120099=DIRECTION('center_axis',(-0.866025403784442,-0.499999999999995,
2.62767925538921E-16));
#120100=DIRECTION('ref_axis',(0.499999999999995,-0.866025403784442,-1.95659843043102E-30));
#120101=DIRECTION('center_axis',(0.866025403784442,0.499999999999995,-2.62767925538921E-16));
#120102=DIRECTION('ref_axis',(-0.499999999999995,0.866025403784442,-1.55538326215048E-32));
#120103=DIRECTION('center_axis',(-0.913545457642603,-0.406736643075795,
2.6945955253847E-16));
#120104=DIRECTION('ref_axis',(0.406736643075795,-0.913545457642603,3.70089423175768E-30));
#120105=DIRECTION('center_axis',(0.913545457642603,0.406736643075795,-2.6945955253847E-16));
#120106=DIRECTION('ref_axis',(-0.406736643075795,0.913545457642603,-1.0068664273239E-32));
#120107=DIRECTION('center_axis',(-0.951056516295156,-0.309016994374942,
2.74741743792088E-16));
#120108=DIRECTION('ref_axis',(0.309016994374942,-0.951056516295155,1.00850339716061E-30));
#120109=DIRECTION('center_axis',(0.951056516295156,0.309016994374942,-2.74741743792088E-16));
#120110=DIRECTION('ref_axis',(-0.309016994374942,0.951056516295156,-2.05892830670188E-33));
#120111=DIRECTION('center_axis',(-0.978147600733807,-0.207911690817753,
2.78556626507032E-16));
#120112=DIRECTION('ref_axis',(0.207911690817753,-0.978147600733807,-2.97094794484635E-30));
#120113=DIRECTION('center_axis',(0.978147600733807,0.207911690817753,-2.78556626507032E-16));
#120114=DIRECTION('ref_axis',(-0.207911690817753,0.978147600733807,2.71817545091438E-33));
#120115=DIRECTION('center_axis',(-0.994521895368274,-0.104528463267647,
2.80862404029962E-16));
#120116=DIRECTION('ref_axis',(0.104528463267647,-0.994521895368274,-2.37338795252393E-30));
#120117=DIRECTION('center_axis',(0.994521895368274,0.104528463267647,-2.80862404029962E-16));
#120118=DIRECTION('ref_axis',(-0.104528463267647,0.994521895368274,5.68888447571522E-33));
#120119=DIRECTION('center_axis',(-1.,0.,2.81633813779821E-16));
#120120=DIRECTION('ref_axis',(2.81633813779821E-16,0.,1.));
#120121=DIRECTION('center_axis',(1.,0.,-2.81633813779821E-16));
#120122=DIRECTION('ref_axis',(-2.81633813779821E-16,0.,-1.));
#120123=DIRECTION('center_axis',(-0.994521895368273,0.104528463267661,2.80862404029962E-16));
#120124=DIRECTION('ref_axis',(-0.104528463267661,-0.994521895368273,-5.04412614481267E-30));
#120125=DIRECTION('center_axis',(0.994521895368273,-0.104528463267661,-2.80862404029962E-16));
#120126=DIRECTION('ref_axis',(0.104528463267661,0.994521895368273,6.74219343631748E-33));
#120127=DIRECTION('center_axis',(-0.978147600733804,0.207911690817766,2.78556626507032E-16));
#120128=DIRECTION('ref_axis',(-0.207911690817766,-0.978147600733804,-4.05861451950599E-30));
#120129=DIRECTION('center_axis',(0.978147600733804,-0.207911690817766,-2.78556626507032E-16));
#120130=DIRECTION('ref_axis',(0.207911690817766,0.978147600733804,1.6755092077588E-33));
#120131=DIRECTION('center_axis',(-0.951056516295151,0.309016994374955,2.74741743792088E-16));
#120132=DIRECTION('ref_axis',(-0.309016994374955,-0.951056516295151,2.69510815298916E-30));
#120133=DIRECTION('center_axis',(0.951056516295151,-0.309016994374955,-2.74741743792088E-16));
#120134=DIRECTION('ref_axis',(0.309016994374954,0.951056516295151,1.52765009372192E-33));
#120135=DIRECTION('center_axis',(-0.913545457642598,0.406736643075807,2.69459552538469E-16));
#120136=DIRECTION('ref_axis',(-0.406736643075807,-0.913545457642598,-2.24713220158703E-30));
#120137=DIRECTION('center_axis',(0.913545457642598,-0.406736643075807,-2.69459552538469E-16));
#120138=DIRECTION('ref_axis',(0.406736643075807,0.913545457642598,4.89387255474364E-33));
#120139=DIRECTION('center_axis',(-0.866025403784435,0.500000000000007,2.6276792553892E-16));
#120140=DIRECTION('ref_axis',(-0.500000000000007,-0.866025403784435,3.04674772188031E-30));
#120141=DIRECTION('center_axis',(0.866025403784435,-0.500000000000007,-2.6276792553892E-16));
#120142=DIRECTION('ref_axis',(0.500000000000007,0.866025403784435,1.00882858511171E-32));
#120143=DIRECTION('center_axis',(-0.809016994374943,0.58778525229248,2.54740177659162E-16));
#120144=DIRECTION('ref_axis',(-0.58778525229248,-0.809016994374943,-2.90930572432627E-30));
#120145=DIRECTION('center_axis',(0.809016994374943,-0.58778525229248,-2.54740177659162E-16));
#120146=DIRECTION('ref_axis',(0.58778525229248,0.809016994374943,-3.19259242211985E-33));
#120147=DIRECTION('center_axis',(-0.743144825477389,0.669130606358864,2.45464262584879E-16));
#120148=DIRECTION('ref_axis',(-0.669130606358864,-0.743144825477389,-5.46633698419621E-31));
#120149=DIRECTION('center_axis',(0.743144825477389,-0.669130606358864,-2.45464262584879E-16));
#120150=DIRECTION('ref_axis',(0.669130606358864,0.743144825477388,3.38071403517698E-33));
#120151=DIRECTION('center_axis',(-0.669130606358852,0.7431448254774,2.35041809182734E-16));
#120152=DIRECTION('ref_axis',(-0.7431448254774,-0.669130606358852,-1.71651837522136E-30));
#120153=DIRECTION('center_axis',(0.669130606358852,-0.7431448254774,-2.35041809182734E-16));
#120154=DIRECTION('ref_axis',(0.7431448254774,0.669130606358852,1.79927205836015E-32));
#120155=DIRECTION('center_axis',(-0.587785252292466,0.809016994374953,2.23587008033241E-16));
#120156=DIRECTION('ref_axis',(-0.809016994374953,-0.587785252292466,-8.24500195267044E-31));
#120157=DIRECTION('center_axis',(0.587785252292466,-0.809016994374953,-2.23587008033241E-16));
#120158=DIRECTION('ref_axis',(0.809016994374953,0.587785252292466,2.52047245046794E-33));
#120159=DIRECTION('center_axis',(-0.499999999999992,0.866025403784443,2.11225360334865E-16));
#120160=DIRECTION('ref_axis',(-0.866025403784443,-0.499999999999992,-8.42158487461594E-31));
#120161=DIRECTION('center_axis',(0.499999999999992,-0.866025403784443,-2.11225360334865E-16));
#120162=DIRECTION('ref_axis',(0.866025403784443,0.499999999999992,1.18398846415295E-32));
#120163=DIRECTION('center_axis',(-0.406736643075792,0.913545457642605,1.98092302886629E-16));
#120164=DIRECTION('ref_axis',(-0.913545457642605,-0.406736643075792,-3.87293527714641E-30));
#120165=DIRECTION('center_axis',(0.406736643075792,-0.913545457642605,-1.98092302886629E-16));
#120166=DIRECTION('ref_axis',(0.913545457642605,0.406736643075792,-1.20511778983704E-32));
#120167=DIRECTION('center_axis',(-0.309016994374938,0.951056516295157,1.84331724214206E-16));
#120168=DIRECTION('ref_axis',(-0.951056516295157,-0.309016994374938,1.32922675182072E-30));
#120169=DIRECTION('center_axis',(0.309016994374938,-0.951056516295157,-1.84331724214206E-16));
#120170=DIRECTION('ref_axis',(0.951056516295157,0.309016994374938,-4.09124323265046E-33));
#120171=DIRECTION('center_axis',(-0.207911690817749,0.978147600733808,1.70094388097117E-16));
#120172=DIRECTION('ref_axis',(-0.978147600733808,-0.207911690817749,-1.14066107666938E-30));
#120173=DIRECTION('center_axis',(0.207911690817749,-0.978147600733808,-1.70094388097117E-16));
#120174=DIRECTION('ref_axis',(0.978147600733808,0.207911690817749,2.34967611901948E-34));
#120175=DIRECTION('center_axis',(-0.104528463267644,0.994521895368275,1.55536281769216E-16));
#120176=DIRECTION('ref_axis',(-0.994521895368274,-0.104528463267644,-7.70551591036319E-31));
#120177=DIRECTION('center_axis',(0.104528463267644,-0.994521895368275,-1.55536281769216E-16));
#120178=DIRECTION('ref_axis',(0.994521895368274,0.104528463267644,1.28454224350036E-33));
#120179=DIRECTION('center_axis',(1.04744440165294E-14,1.,1.40816906889909E-16));
#120180=DIRECTION('ref_axis',(-1.,1.04744440165294E-14,1.47497880779919E-30));
#120181=DIRECTION('center_axis',(-1.04744440165294E-14,-1.,-1.40816906889909E-16));
#120182=DIRECTION('ref_axis',(1.,-1.04744440165294E-14,5.25486924121806E-46));
#120183=DIRECTION('center_axis',(0.104528463267664,0.994521895368272,1.26097532010602E-16));
#120184=DIRECTION('ref_axis',(-0.994521895368272,0.104528463267664,-1.87870457210236E-30));
#120185=DIRECTION('center_axis',(-0.104528463267664,-0.994521895368272,
-1.26097532010602E-16));
#120186=DIRECTION('ref_axis',(0.994521895368272,-0.104528463267664,1.52293880083755E-33));
#120187=DIRECTION('center_axis',(0.20791169081777,0.978147600733803,1.11539425682701E-16));
#120188=DIRECTION('ref_axis',(-0.978147600733803,0.20791169081777,-1.23488624019268E-30));
#120189=DIRECTION('center_axis',(-0.20791169081777,-0.978147600733803,-1.11539425682701E-16));
#120190=DIRECTION('ref_axis',(0.978147600733803,-0.20791169081777,6.98244303227918E-33));
#120191=DIRECTION('center_axis',(0.309016994374957,0.95105651629515,9.73020895656121E-17));
#120192=DIRECTION('ref_axis',(-0.95105651629515,0.309016994374957,1.25555458542293E-30));
#120193=DIRECTION('center_axis',(-0.309016994374957,-0.95105651629515,-9.73020895656121E-17));
#120194=DIRECTION('ref_axis',(0.95105651629515,-0.309016994374957,-1.05677412542168E-33));
#120195=DIRECTION('center_axis',(0.40673664307581,0.913545457642596,8.35415108931894E-17));
#120196=DIRECTION('ref_axis',(-0.913545457642597,0.40673664307581,-3.95491880831218E-31));
#120197=DIRECTION('center_axis',(-0.40673664307581,-0.913545457642596,-8.35415108931894E-17));
#120198=DIRECTION('ref_axis',(0.913545457642596,-0.40673664307581,1.14994985725664E-33));
#120199=DIRECTION('center_axis',(0.50000000000001,0.866025403784433,7.04084534449538E-17));
#120200=DIRECTION('ref_axis',(-0.866025403784433,0.50000000000001,-1.35169061292236E-30));
#120201=DIRECTION('center_axis',(-0.50000000000001,-0.866025403784433,-7.04084534449538E-17));
#120202=DIRECTION('ref_axis',(0.866025403784433,-0.50000000000001,3.15276542668096E-33));
#120203=DIRECTION('center_axis',(0.587785252292482,0.809016994374941,5.80468057465775E-17));
#120204=DIRECTION('ref_axis',(-0.809016994374941,0.587785252292482,-4.87668228627595E-31));
#120205=DIRECTION('center_axis',(-0.587785252292482,-0.809016994374941,
-5.80468057465775E-17));
#120206=DIRECTION('ref_axis',(0.809016994374941,-0.587785252292482,-7.07752156141996E-33));
#120207=DIRECTION('center_axis',(0.669130606358867,0.743144825477386,4.65920045970846E-17));
#120208=DIRECTION('ref_axis',(-0.743144825477386,0.669130606358867,6.2996129283645E-32));
#120209=DIRECTION('center_axis',(-0.669130606358867,-0.743144825477386,
-4.65920045970846E-17));
#120210=DIRECTION('ref_axis',(0.743144825477386,-0.669130606358867,-1.70435726196324E-33));
#120211=DIRECTION('center_axis',(0.743144825477402,0.66913060635885,3.61695511949404E-17));
#120212=DIRECTION('ref_axis',(-0.66913060635885,0.743144825477402,-1.54743219885707E-31));
#120213=DIRECTION('center_axis',(-0.743144825477402,-0.66913060635885,-3.61695511949404E-17));
#120214=DIRECTION('ref_axis',(0.66913060635885,-0.743144825477402,-1.64364935203297E-33));
#120215=DIRECTION('center_axis',(0.809016994374955,0.587785252292463,2.68936361206573E-17));
#120216=DIRECTION('ref_axis',(-0.587785252292463,0.809016994374955,-6.32658501432878E-31));
#120217=DIRECTION('center_axis',(-0.809016994374955,-0.587785252292463,
-2.68936361206573E-17));
#120218=DIRECTION('ref_axis',(0.587785252292463,-0.809016994374955,5.77490301261619E-34));
#120219=DIRECTION('center_axis',(0.866025403784445,0.499999999999989,1.88658882408992E-17));
#120220=DIRECTION('ref_axis',(-0.499999999999989,0.866025403784445,-9.02647084236321E-33));
#120221=DIRECTION('center_axis',(-0.866025403784445,-0.499999999999989,
-1.88658882408992E-17));
#120222=DIRECTION('ref_axis',(0.499999999999989,-0.866025403784445,-2.17992890695449E-34));
#120223=DIRECTION('center_axis',(0.913545457642606,0.406736643075789,1.2174261241351E-17));
#120224=DIRECTION('ref_axis',(-0.406736643075789,0.913545457642606,-1.9369316171316E-31));
#120225=DIRECTION('center_axis',(-0.913545457642606,-0.406736643075789,
-1.2174261241351E-17));
#120226=DIRECTION('ref_axis',(0.406736643075789,-0.913545457642606,-6.72158879142273E-34));
#120227=DIRECTION('center_axis',(0.951056516295158,0.309016994374935,6.89206998773264E-18));
#120228=DIRECTION('ref_axis',(-0.309016994374935,0.951056516295158,7.38462266190487E-32));
#120229=DIRECTION('center_axis',(-0.951056516295158,-0.309016994374935,
-6.89206998773264E-18));
#120230=DIRECTION('ref_axis',(0.309016994374935,-0.951056516295158,1.7074848336093E-34));
#120231=DIRECTION('center_axis',(0.978147600733808,0.207911690817747,3.07718727278847E-18));
#120232=DIRECTION('ref_axis',(-0.207911690817747,0.978147600733808,-1.89718420003736E-32));
#120233=DIRECTION('center_axis',(-0.978147600733808,-0.207911690817747,
-3.07718727278847E-18));
#120234=DIRECTION('ref_axis',(0.207911690817747,-0.978147600733808,5.10419938729071E-35));
#120235=DIRECTION('center_axis',(0.994521895368275,0.10452846326764,7.71409749858844E-19));
#120236=DIRECTION('ref_axis',(-0.10452846326764,0.994521895368275,-1.11530674608181E-33));
#120237=DIRECTION('center_axis',(-0.994521895368275,-0.10452846326764,-7.71409749858844E-19));
#120238=DIRECTION('ref_axis',(0.10452846326764,-0.994521895368275,2.19054274915971E-35));
#120239=DIRECTION('center_axis',(-0.497265934575652,0.0522647557772525,
0.866022508722578));
#120240=DIRECTION('ref_axis',(0.104528463268683,0.994521895368165,5.94450124796257E-13));
#120241=DIRECTION('center_axis',(-0.86127722484323,0.0904936763723186,0.500012436348305));
#120242=DIRECTION('ref_axis',(0.49716964624231,-0.0532497882904349,0.866017784403023));
#120243=DIRECTION('center_axis',(0.497265943181924,-0.0522647566817888,
-0.866022503726309));
#120244=DIRECTION('ref_axis',(-0.867207748104374,9.14067291315517E-16,-0.497946504785143));
#120245=DIRECTION('center_axis',(0.994521895368276,-0.104528463267628,0.));
#120246=DIRECTION('ref_axis',(0.104528463267628,0.994521895368276,0.));
#120247=DIRECTION('center_axis',(-0.994521895368273,0.104528463267654,1.40045497140051E-16));
#120248=DIRECTION('ref_axis',(-0.104528463267654,-0.994521895368273,1.88774370219345E-33));
#120249=DIRECTION('center_axis',(-0.994521895368276,0.104528463267629,-1.42777936329238E-15));
#120250=DIRECTION('ref_axis',(-0.104528463267629,-0.994521895368276,-1.03141617847887E-30));
#120251=DIRECTION('center_axis',(-0.994521895368273,0.104528463267654,1.40045497140051E-16));
#120252=DIRECTION('ref_axis',(-0.104528463267654,-0.994521895368273,1.88774370219345E-33));
#120253=DIRECTION('center_axis',(0.994521895368276,-0.104528463267628,0.));
#120254=DIRECTION('ref_axis',(0.104528463267628,0.994521895368276,0.));
#120255=DIRECTION('center_axis',(-0.527021232978597,0.0553921636609763,
-0.848045003637587));
#120256=DIRECTION('ref_axis',(-0.849349030019387,-1.18520091513627E-15,
0.527831625809904));
#120257=DIRECTION('center_axis',(0.497266077958583,-0.0522647708474063,
0.866022425483288));
#120258=DIRECTION('ref_axis',(0.867207670398076,2.13898382432694E-16,-0.497946640115929));
#120259=DIRECTION('center_axis',(0.52702120261152,-0.0553921822138802,0.848045021297509));
#120260=DIRECTION('ref_axis',(0.842941044395424,-0.0929299148179921,-0.529919264233215));
#120261=DIRECTION('center_axis',(-0.527021177161361,0.0553921577943484,
-0.84804503870864));
#120262=DIRECTION('ref_axis',(-0.84934906486751,-4.67755375184424E-16,0.527831569734783));
#120263=DIRECTION('center_axis',(0.497266090634776,-0.0522647827596761,
0.866022417485766));
#120264=DIRECTION('ref_axis',(0.86079389248998,-0.0950466972174585,-0.500000000000001));
#120265=DIRECTION('center_axis',(0.861296695145091,-0.0904912830030048,
0.499979330205374));
#120266=DIRECTION('ref_axis',(0.497340894869929,-0.0513033469932807,-0.866036951219326));
#120267=DIRECTION('center_axis',(-0.104769627595161,-0.994496518411991,
6.79203329632462E-15));
#120268=DIRECTION('ref_axis',(0.994496518411991,-0.104769627595161,3.19732566850161E-29));
#120269=DIRECTION('center_axis',(-0.994521895368273,0.104528463267654,1.40045497140051E-16));
#120270=DIRECTION('ref_axis',(-0.104528463267654,-0.994521895368273,1.88774370219345E-33));
#120271=DIRECTION('center_axis',(0.994521895368276,-0.104528463267627,0.));
#120272=DIRECTION('ref_axis',(0.104528463267627,0.994521895368276,0.));
#120273=DIRECTION('center_axis',(-7.71409749859041E-19,-1.47193748793066E-17,
-1.));
#120274=DIRECTION('ref_axis',(0.,1.,0.));
#120275=DIRECTION('center_axis',(-0.104287292793436,-0.994547213842468,
0.));
#120276=DIRECTION('ref_axis',(0.994547213842468,-0.104287292793436,0.));
#120277=DIRECTION('center_axis',(0.52702169399903,-0.0553922121162226,-0.848044713969295));
#120278=DIRECTION('ref_axis',(-0.849348742192381,8.56035801599993E-16,-0.527832088960325));
#120279=DIRECTION('center_axis',(0.52702117716142,-0.0553921577944011,0.8480450387086));
#120280=DIRECTION('ref_axis',(0.849349064867473,2.16233168370015E-16,-0.527831569734843));
#120281=DIRECTION('center_axis',(0.527021729069701,-0.0553921904551721,
-0.848044693589295));
#120282=DIRECTION('ref_axis',(-0.842916495802325,0.0931523188055466,-0.529919264233222));
#120283=DIRECTION('center_axis',(0.527021758969982,-0.0553922189448986,
-0.848044673146731));
#120284=DIRECTION('ref_axis',(-0.849348701629304,3.9911212985723E-16,-0.527832154231452));
#120285=DIRECTION('center_axis',(-0.527021202762352,0.0553921822934361,
-0.848045021198577));
#120286=DIRECTION('ref_axis',(0.843841975851001,-0.0843581246018643,-0.529919264233275));
#120287=DIRECTION('center_axis',(0.527021232978612,-0.0553921636609779,
0.848045003637578));
#120288=DIRECTION('ref_axis',(0.849349030019378,-4.13967457904561E-16,-0.527831625809918));
#120289=DIRECTION('center_axis',(-0.10478522557409,-0.994494875050338,0.));
#120290=DIRECTION('ref_axis',(0.994494875050338,-0.10478522557409,0.));
#120291=DIRECTION('center_axis',(0.994521895368276,-0.104528463267629,0.));
#120292=DIRECTION('ref_axis',(0.104528463267629,0.994521895368276,0.));
#120293=DIRECTION('center_axis',(-7.71409749859041E-19,-1.47193748793066E-17,
-1.));
#120294=DIRECTION('ref_axis',(0.,1.,0.));
#120295=DIRECTION('center_axis',(-0.104271693993672,-0.994548849394382,
6.79239069704775E-15));
#120296=DIRECTION('ref_axis',(0.994548849394382,-0.104271693993672,1.8061767832882E-30));
#120297=DIRECTION('center_axis',(0.994521895368273,-0.104528463267654,-1.40045497140051E-16));
#120298=DIRECTION('ref_axis',(0.104528463267654,0.994521895368273,-3.47023617217699E-30));
#120299=DIRECTION('center_axis',(0.861270944309928,-0.0905534316539297,
-0.500012436348519));
#120300=DIRECTION('ref_axis',(0.497376550150566,-0.0512812291022556,0.866017784402886));
#120301=DIRECTION('center_axis',(-0.527021758969975,0.0553922189448978,
0.848044673146736));
#120302=DIRECTION('ref_axis',(0.849348701629309,-8.88691521652723E-16,0.527832154231445));
#120303=DIRECTION('center_axis',(-0.497265930897887,0.0522647452181895,
0.866022511471576));
#120304=DIRECTION('ref_axis',(-0.861737632556526,0.0860712067763655,-0.499999999999934));
#120305=DIRECTION('center_axis',(0.497265943181814,-0.0522647566817776,
-0.866022503726373));
#120306=DIRECTION('ref_axis',(-0.867207748104437,-2.31772315575697E-16,
-0.497946504785033));
#120307=DIRECTION('center_axis',(-0.52702172888514,0.055392190353939,0.848044693710603));
#120308=DIRECTION('ref_axis',(-0.843864204095268,0.0841354767099045,-0.5299192642332));
#120309=DIRECTION('center_axis',(-0.527021693998978,0.0553922121161999,
0.848044713969329));
#120310=DIRECTION('ref_axis',(0.849348742192414,-1.18056289443676E-16,0.527832088960272));
#120311=DIRECTION('center_axis',(0.994521895368276,-0.104528463267629,0.));
#120312=DIRECTION('ref_axis',(0.104528463267629,0.994521895368276,0.));
#120313=DIRECTION('center_axis',(-0.994521895368276,0.104528463267629,0.));
#120314=DIRECTION('ref_axis',(-0.104528463267629,-0.994521895368276,0.));
#120315=DIRECTION('center_axis',(0.994521895368273,-0.104528463267654,-1.40045497140051E-16));
#120316=DIRECTION('ref_axis',(0.104528463267654,0.994521895368273,-3.47023617217699E-30));
#120317=DIRECTION('center_axis',(0.994521895368276,-0.104528463267629,-7.13889681646191E-16));
#120318=DIRECTION('ref_axis',(0.104528463267629,0.994521895368276,-5.15708089239434E-31));
#120319=DIRECTION('center_axis',(0.994521895368273,-0.104528463267654,-1.40045497140051E-16));
#120320=DIRECTION('ref_axis',(0.104528463267654,0.994521895368273,-3.47023617217699E-30));
#120321=DIRECTION('center_axis',(-0.861289491529685,0.0905598208268781,
-0.4999793302051));
#120322=DIRECTION('ref_axis',(0.497139368681443,-0.0532207405949754,-0.866036951219484));
#120323=DIRECTION('center_axis',(0.497266077958573,-0.0522647708473857,
0.866022425483295));
#120324=DIRECTION('ref_axis',(0.867207670398082,-3.99694090177787E-16,-0.497946640115919));
#120325=DIRECTION('center_axis',(0.497266086881316,-0.0522647717852188,
0.866022420303298));
#120326=DIRECTION('ref_axis',(-0.104528463263483,-0.994521895368712,-2.44773579649901E-12));
#120327=DIRECTION('center_axis',(-0.489078705154303,0.103956887953619,0.866022508721101));
#120328=DIRECTION('ref_axis',(0.207911690815745,0.978147600734234,-1.18890024958885E-12));
#120329=DIRECTION('center_axis',(-0.84709989316159,0.180025927305589,0.500012436348723));
#120330=DIRECTION('ref_axis',(0.488879980351047,-0.104926459533017,0.866017784402737));
#120331=DIRECTION('center_axis',(0.489078713616375,-0.103956889752293,-0.866022503726307));
#120332=DIRECTION('ref_axis',(-0.8707403454847,1.23854993518449E-15,-0.491743073916843));
#120333=DIRECTION('center_axis',(0.978147600733807,-0.207911690817754,0.));
#120334=DIRECTION('ref_axis',(0.207911690817754,0.978147600733807,0.));
#120335=DIRECTION('center_axis',(-0.978147600733806,0.20791169081776,1.37739719617122E-16));
#120336=DIRECTION('ref_axis',(-0.20791169081776,-0.978147600733805,-5.54372792423441E-34));
#120337=DIRECTION('center_axis',(-0.978147600733806,0.207911690817757,0.));
#120338=DIRECTION('ref_axis',(-0.207911690817757,-0.978147600733806,0.));
#120339=DIRECTION('center_axis',(-0.978147600733806,0.20791169081776,1.37739719617122E-16));
#120340=DIRECTION('ref_axis',(-0.20791169081776,-0.978147600733805,-5.54372792423441E-34));
#120341=DIRECTION('center_axis',(0.978147600733806,-0.207911690817757,0.));
#120342=DIRECTION('ref_axis',(0.207911690817757,0.978147600733806,0.));
#120343=DIRECTION('center_axis',(-0.518344097776643,0.110177439185352,-0.848045003637588));
#120344=DIRECTION('ref_axis',(-0.853239582811875,-1.68392254271072E-15,
0.521519140898028));
#120345=DIRECTION('center_axis',(0.489078846174041,-0.103956917928293,0.866022425483266));
#120346=DIRECTION('ref_axis',(0.870740269393754,4.19086328667376E-16,-0.491743208652741));
#120347=DIRECTION('center_axis',(0.518344065636325,-0.110177454463846,0.848045021297497));
#120348=DIRECTION('ref_axis',(0.828609503966741,-0.180532167024357,-0.529919264233224));
#120349=DIRECTION('center_axis',(-0.518344042878402,0.11017742751637,-0.848045038708646));
#120350=DIRECTION('ref_axis',(-0.853239616987301,8.06953644704382E-16,0.521519084984782));
#120351=DIRECTION('center_axis',(0.48907885753683,-0.103956931094349,0.866022417485779));
#120352=DIRECTION('ref_axis',(0.846143288282877,-0.18450348423235,-0.499999999999963));
#120353=DIRECTION('center_axis',(0.847119506978939,-0.180025582247288,0.499979330205044));
#120354=DIRECTION('ref_axis',(0.489253749388313,-0.103008581350701,-0.866036951219516));
#120355=DIRECTION('center_axis',(-0.208148881407599,-0.978097154258597,
0.));
#120356=DIRECTION('ref_axis',(0.978097154258597,-0.2081488814076,0.));
#120357=DIRECTION('center_axis',(-0.978147600733806,0.20791169081776,1.37739719617122E-16));
#120358=DIRECTION('ref_axis',(-0.20791169081776,-0.978147600733805,-5.54372792423441E-34));
#120359=DIRECTION('center_axis',(0.978147600733806,-0.207911690817757,0.));
#120360=DIRECTION('ref_axis',(0.207911690817757,0.978147600733806,0.));
#120361=DIRECTION('center_axis',(-3.07718727278886E-18,-2.92774812072083E-17,
-1.));
#120362=DIRECTION('ref_axis',(0.,1.,0.));
#120363=DIRECTION('center_axis',(-0.20767448800182,-0.978197989689808,0.));
#120364=DIRECTION('ref_axis',(0.978197989689808,-0.20767448800182,0.));
#120365=DIRECTION('center_axis',(0.518344551206617,-0.11017753556485,-0.848044713969297));
#120366=DIRECTION('ref_axis',(-0.85323930054102,-8.4671885596076E-16,-0.521519602711414));
#120367=DIRECTION('center_axis',(0.518344042878406,-0.110177427516371,0.848045038708643));
#120368=DIRECTION('ref_axis',(0.853239616987298,-2.86146343343731E-16,-0.521519084984786));
#120369=DIRECTION('center_axis',(0.518344588349843,-0.110177517686205,-0.848044693589281));
#120370=DIRECTION('ref_axis',(-0.828561842307295,0.18075078662857,-0.529919264233236));
#120371=DIRECTION('center_axis',(0.518344615107834,-0.110177549147491,-0.848044673146742));
#120372=DIRECTION('ref_axis',(-0.853239260760976,-2.80784050022121E-15,
-0.521519667794095));
#120373=DIRECTION('center_axis',(-0.518344065777496,0.110177454561188,-0.848045021198564));
#120374=DIRECTION('ref_axis',(0.83040149609203,-0.172101506915709,-0.529919264233205));
#120375=DIRECTION('center_axis',(0.518344097776693,-0.110177439185362,0.848045003637556));
#120376=DIRECTION('ref_axis',(0.853239582811844,4.32157940244689E-18,-0.521519140898079));
#120377=DIRECTION('center_axis',(-0.208164222161104,-0.978093889466682,
0.));
#120378=DIRECTION('ref_axis',(0.978093889466682,-0.208164222161104,0.));
#120379=DIRECTION('center_axis',(0.978147600733806,-0.207911690817757,0.));
#120380=DIRECTION('ref_axis',(0.207911690817757,0.978147600733806,0.));
#120381=DIRECTION('center_axis',(-3.07718727278886E-18,-2.92774812072083E-17,
-1.));
#120382=DIRECTION('ref_axis',(0.,1.,0.));
#120383=DIRECTION('center_axis',(-0.207659145615656,-0.978201246800563,
0.));
#120384=DIRECTION('ref_axis',(0.978201246800563,-0.207659145615656,0.));
#120385=DIRECTION('center_axis',(0.978147600733806,-0.20791169081776,-1.37739719617122E-16));
#120386=DIRECTION('ref_axis',(0.20791169081776,0.978147600733806,-3.77399900463914E-31));
#120387=DIRECTION('center_axis',(0.847087400906584,-0.180084698746639,-0.500012436347998));
#120388=DIRECTION('ref_axis',(0.489291521293116,-0.10299031162228,0.866017784403192));
#120389=DIRECTION('center_axis',(-0.518344615107832,0.110177549147519,0.848044673146739));
#120390=DIRECTION('ref_axis',(0.853239260760976,2.80072453551802E-15,0.521519667794095));
#120391=DIRECTION('center_axis',(-0.489078702597035,0.103956877071927,0.866022511471528));
#120392=DIRECTION('ref_axis',(-0.848020052664818,0.175675810168452,-0.500000000000017));
#120393=DIRECTION('center_axis',(0.489078713616259,-0.103956889752268,-0.866022503726375));
#120394=DIRECTION('ref_axis',(-0.870740345484766,2.53322569711339E-15,-0.491743073916726));
#120395=DIRECTION('center_axis',(-0.518344588176244,0.11017751756908,0.848044693710606));
#120396=DIRECTION('ref_axis',(-0.830446875604741,0.171882402219908,-0.529919264233183));
#120397=DIRECTION('center_axis',(-0.518344551206558,0.110177535564884,0.848044713969329));
#120398=DIRECTION('ref_axis',(0.853239300541055,1.68070280509443E-15,0.521519602711356));
#120399=DIRECTION('center_axis',(0.978147600733806,-0.207911690817757,0.));
#120400=DIRECTION('ref_axis',(0.207911690817757,0.978147600733806,0.));
#120401=DIRECTION('center_axis',(-0.978147600733806,0.207911690817757,0.));
#120402=DIRECTION('ref_axis',(-0.207911690817757,-0.978147600733806,0.));
#120403=DIRECTION('center_axis',(0.978147600733806,-0.20791169081776,-1.37739719617122E-16));
#120404=DIRECTION('ref_axis',(0.20791169081776,0.978147600733806,-3.77399900463914E-31));
#120405=DIRECTION('center_axis',(0.978147600733806,-0.207911690817757,-2.83991567709912E-15));
#120406=DIRECTION('ref_axis',(0.207911690817757,0.978147600733806,-3.75217731718872E-32));
#120407=DIRECTION('center_axis',(0.978147600733806,-0.20791169081776,-1.37739719617122E-16));
#120408=DIRECTION('ref_axis',(0.20791169081776,0.978147600733806,-3.77399900463914E-31));
#120409=DIRECTION('center_axis',(-0.847105178672012,0.18009299163106,-0.499979330205193));
#120410=DIRECTION('ref_axis',(0.488852904976213,-0.104894406041813,-0.866036951219434));
#120411=DIRECTION('center_axis',(0.489078846174021,-0.10395691792829,0.866022425483278));
#120412=DIRECTION('ref_axis',(0.870740269393765,2.98920110677976E-15,-0.491743208652721));
#120413=DIRECTION('center_axis',(0.489078854952772,-0.103956919794272,0.866022420301561));
#120414=DIRECTION('ref_axis',(-0.207911690815506,-0.978147600734285,-1.36373851518786E-12));
#120415=DIRECTION('center_axis',(-0.475533027087639,0.154510046710004,0.866022508722804));
#120416=DIRECTION('ref_axis',(0.309016994373617,0.951056516295586,-7.69288396791546E-13));
#120417=DIRECTION('center_axis',(-0.823641557784419,0.267585776505498,0.500012436347742));
#120418=DIRECTION('ref_axis',(0.475234043097329,-0.155453534467842,0.866017784403312));
#120419=DIRECTION('center_axis',(0.475533035318149,-0.154510049384271,-0.866022503726305));
#120420=DIRECTION('ref_axis',(-0.876548788012431,-5.39585338525745E-15,
-0.481313018974075));
#120421=DIRECTION('center_axis',(0.951056516295146,-0.309016994374972,0.));
#120422=DIRECTION('ref_axis',(0.309016994374972,0.951056516295146,0.));
#120423=DIRECTION('center_axis',(-0.951056516295153,0.309016994374948,1.33924836902177E-16));
#120424=DIRECTION('ref_axis',(-0.309016994374948,-0.951056516295153,2.44548634228625E-33));
#120425=DIRECTION('center_axis',(-0.951056516295148,0.309016994374964,0.));
#120426=DIRECTION('ref_axis',(-0.309016994374964,-0.951056516295148,0.));
#120427=DIRECTION('center_axis',(-0.951056516295153,0.309016994374948,1.33924836902177E-16));
#120428=DIRECTION('ref_axis',(-0.309016994374948,-0.951056516295153,-9.88046530179205E-33));
#120429=DIRECTION('center_axis',(0.951056516295165,-0.309016994374914,0.));
#120430=DIRECTION('ref_axis',(0.309016994374914,0.951056516295164,0.));
#120431=DIRECTION('center_axis',(-0.503987876168977,0.163755587629901,-0.848045003637584));
#120432=DIRECTION('ref_axis',(-0.859649462041493,-1.98479274860628E-15,
0.510884333691857));
#120433=DIRECTION('center_axis',(0.475533164204456,-0.154510091261994,0.86602242548326));
#120434=DIRECTION('ref_axis',(0.87654871462881,-1.83225743718063E-16,-0.481313152617483));
#120435=DIRECTION('center_axis',(0.503987842609227,-0.163755599460403,0.848045021297491));
#120436=DIRECTION('ref_axis',(0.805199544420487,-0.266156471008179,-0.529919264233254));
#120437=DIRECTION('center_axis',(-0.503987822791217,0.163755570286415,-0.848045038708641));
#120438=DIRECTION('ref_axis',(-0.859649495083695,-2.20730751304904E-15,
0.510884278092748));
#120439=DIRECTION('center_axis',(0.475533174128361,-0.154510105545038,0.866022417485753));
#120440=DIRECTION('ref_axis',(0.822222161142858,-0.271938812466216,-0.500000000000033));
#120441=DIRECTION('center_axis',(0.823661100222795,-0.267587483540072,0.499979330205226));
#120442=DIRECTION('ref_axis',(0.475806237441931,-0.153585232147895,-0.866036951219421));
#120443=DIRECTION('center_axis',(-0.309247612517368,-0.950981553003163,
0.));
#120444=DIRECTION('ref_axis',(0.950981553003163,-0.309247612517368,0.));
#120445=DIRECTION('center_axis',(-0.951056516295153,0.309016994374948,1.33924836902177E-16));
#120446=DIRECTION('ref_axis',(-0.309016994374948,-0.951056516295153,2.44548634228625E-33));
#120447=DIRECTION('center_axis',(0.951056516295165,-0.309016994374914,0.));
#120448=DIRECTION('ref_axis',(0.309016994374914,0.951056516295164,0.));
#120449=DIRECTION('center_axis',(-6.89206998773325E-18,-4.35148173242971E-17,
-1.));
#120450=DIRECTION('ref_axis',(0.,1.,0.));
#120451=DIRECTION('center_axis',(-0.308786358061007,-0.95113142366101,0.));
#120452=DIRECTION('ref_axis',(0.95113142366101,-0.308786358061007,0.));
#120453=DIRECTION('center_axis',(0.503988317040591,-0.163755730877772,-0.848044713969304));
#120454=DIRECTION('ref_axis',(-0.859649189130459,-2.98011051076997E-15,
-0.510884792910637));
#120455=DIRECTION('center_axis',(0.503987822791257,-0.163755570286477,0.848045038708605));
#120456=DIRECTION('ref_axis',(0.859649495083668,3.24166635856024E-15,-0.510884278092793));
#120457=DIRECTION('center_axis',(0.50398835585061,-0.163755716975207,-0.84804469358928));
#120458=DIRECTION('ref_axis',(-0.80512929187801,0.266368911013597,-0.529919264233189));
#120459=DIRECTION('center_axis',(0.503988379172007,-0.163755751065444,-0.848044673146743));
#120460=DIRECTION('ref_axis',(-0.859649150669465,-1.48397689224786E-15,
-0.510884857627692));
#120461=DIRECTION('center_axis',(-0.503987842737447,0.163755599578063,-0.84804502119857));
#120462=DIRECTION('ref_axis',(0.807862963766411,-0.257959309134419,-0.529919264233189));
#120463=DIRECTION('center_axis',(0.503987876169007,-0.163755587629911,0.848045003637564));
#120464=DIRECTION('ref_axis',(0.859649462041474,1.63915119993853E-16,-0.510884333691888));
#120465=DIRECTION('center_axis',(-0.309262527968962,-0.950976702550723,
-1.68971643309507E-14));
#120466=DIRECTION('ref_axis',(0.950976702550723,-0.309262527968962,2.40620234987808E-29));
#120467=DIRECTION('center_axis',(0.951056516295148,-0.309016994374964,-5.19628367180436E-14));
#120468=DIRECTION('ref_axis',(0.309016994374964,0.951056516295148,4.43497354731716E-28));
#120469=DIRECTION('center_axis',(-6.89206998773325E-18,-4.35148173242971E-17,
-1.));
#120470=DIRECTION('ref_axis',(0.,1.,0.));
#120471=DIRECTION('center_axis',(-0.308771440182806,-0.951136266645025,
0.));
#120472=DIRECTION('ref_axis',(0.951136266645025,-0.308771440182806,0.));
#120473=DIRECTION('center_axis',(0.951056516295153,-0.309016994374948,-1.33924836902177E-16));
#120474=DIRECTION('ref_axis',(0.309016994374948,0.951056516295153,2.18771486896698E-30));
#120475=DIRECTION('center_axis',(0.823622990673383,-0.267642920194819,-0.500012436349159));
#120476=DIRECTION('ref_axis',(0.475845712144249,-0.153571010716547,0.866017784402509));
#120477=DIRECTION('center_axis',(-0.503988379172001,0.163755751065515,0.848044673146732));
#120478=DIRECTION('ref_axis',(0.859649150669465,1.54206212768985E-15,0.510884857627692));
#120479=DIRECTION('center_axis',(-0.475533025685691,0.154510035618062,0.866022511471565));
#120480=DIRECTION('ref_axis',(-0.825011387615653,0.26335567262647,-0.499999999999955));
#120481=DIRECTION('center_axis',(0.475533035318008,-0.154510049384248,-0.866022503726387));
#120482=DIRECTION('ref_axis',(-0.87654878801251,1.1206608856956E-15,-0.481313018973931));
#120483=DIRECTION('center_axis',(-0.503988355688897,0.163755716844529,0.848044693710618));
#120484=DIRECTION('ref_axis',(-0.807930997359887,0.257746148176091,-0.529919264233191));
#120485=DIRECTION('center_axis',(-0.50398831704056,0.163755730877767,0.848044713969324));
#120486=DIRECTION('ref_axis',(0.859649189130477,-3.08352198662565E-15,0.510884792910606));
#120487=DIRECTION('center_axis',(0.951056516295148,-0.309016994374964,-5.19628367180436E-14));
#120488=DIRECTION('ref_axis',(0.309016994374964,0.951056516295148,4.43497354731716E-28));
#120489=DIRECTION('center_axis',(-0.951056516295148,0.309016994374964,0.));
#120490=DIRECTION('ref_axis',(-0.309016994374964,-0.951056516295148,0.));
#120491=DIRECTION('center_axis',(0.951056516295153,-0.309016994374948,-1.33924836902177E-16));
#120492=DIRECTION('ref_axis',(0.309016994374948,0.951056516295153,2.18771486896698E-30));
#120493=DIRECTION('center_axis',(0.951056516295148,-0.309016994374964,1.68837491218278E-14));
#120494=DIRECTION('ref_axis',(0.309016994374964,0.951056516295148,-1.43380940262431E-28));
#120495=DIRECTION('center_axis',(0.951056516295153,-0.309016994374948,-1.33924836902177E-16));
#120496=DIRECTION('ref_axis',(0.309016994374948,0.951056516295153,2.18771486896698E-30));
#120497=DIRECTION('center_axis',(-0.823639804208726,0.267653025932271,-0.499979330205069));
#120498=DIRECTION('ref_axis',(0.475210466544137,-0.155418826431445,-0.866036951219506));
#120499=DIRECTION('center_axis',(0.475533164204417,-0.154510091261981,0.866022425483284));
#120500=DIRECTION('ref_axis',(0.876548714628833,4.04293055823746E-15,-0.481313152617442));
#120501=DIRECTION('center_axis',(0.475533172741623,-0.154510094035866,0.866022420300602));
#120502=DIRECTION('ref_axis',(-0.309016994371688,-0.951056516296213,-1.95818863719932E-12));
#120503=DIRECTION('center_axis',(-0.456777309666909,0.203370361061781,0.866022508723105));
#120504=DIRECTION('ref_axis',(0.406736643080227,0.91354545764063,2.76244469758968E-12));
#120505=DIRECTION('center_axis',(-0.791159233140786,0.352213899941099,0.500012436349702));
#120506=DIRECTION('ref_axis',(0.456381342218119,-0.204277427960925,0.866017784402178));
#120507=DIRECTION('center_axis',(0.456777317573273,-0.203370364581912,-0.86602250372631));
#120508=DIRECTION('ref_axis',(-0.884507036382098,5.88362210846088E-15,-0.466526850878444));
#120509=DIRECTION('center_axis',(0.913545457642594,-0.406736643075817,6.10247733350035E-14));
#120510=DIRECTION('ref_axis',(0.406736643075817,0.913545457642593,6.78980940604894E-28));
#120511=DIRECTION('center_axis',(-0.913545457642601,0.406736643075801,1.28642645648559E-16));
#120512=DIRECTION('ref_axis',(-0.406736643075801,-0.9135454576426,-7.47472011570615E-33));
#120513=DIRECTION('center_axis',(-0.913545457642598,0.406736643075807,0.));
#120514=DIRECTION('ref_axis',(-0.406736643075807,-0.913545457642598,0.));
#120515=DIRECTION('center_axis',(-0.913545457642601,0.406736643075801,1.28642645648559E-16));
#120516=DIRECTION('ref_axis',(-0.406736643075801,-0.9135454576426,-7.47472011570615E-33));
#120517=DIRECTION('center_axis',(0.913545457642594,-0.406736643075817,0.));
#120518=DIRECTION('ref_axis',(0.406736643075817,0.913545457642593,0.));
#120519=DIRECTION('center_axis',(-0.48410985792377,0.215539595588306,-0.848045003637576));
#120520=DIRECTION('ref_axis',(-0.868458021515995,5.72874239606451E-16,0.495762710240013));
#120521=DIRECTION('center_axis',(0.456777441376059,-0.203370419702482,0.8660224254833));
#120522=DIRECTION('ref_axis',(0.884506966812066,3.90936356972174E-15,-0.466526982779044));
#120523=DIRECTION('center_axis',(0.48410982330659,-0.215539603856382,0.848045021297511));
#120524=DIRECTION('ref_axis',(0.77296765014953,-0.348864709044782,-0.52991926423316));
#120525=DIRECTION('center_axis',(-0.484109806651296,0.21553957276033,-0.84804503870864));
#120526=DIRECTION('ref_axis',(-0.868458052949953,-3.34246373676304E-15,
0.495762655175213));
#120527=DIRECTION('center_axis',(0.456777449752137,-0.20337043494584,0.866022417485756));
#120528=DIRECTION('ref_axis',(0.789292595943427,-0.356394722167529,-0.500000000000016));
#120529=DIRECTION('center_axis',(0.791178490090755,-0.352217640366503,0.499979330205125));
#120530=DIRECTION('ref_axis',(0.457145692791346,-0.202479170989976,-0.86603695121948));
#120531=DIRECTION('center_axis',(-0.406958162070229,-0.913446798847323,
0.));
#120532=DIRECTION('ref_axis',(0.913446798847323,-0.406958162070229,0.));
#120533=DIRECTION('center_axis',(-0.913545457642601,0.406736643075801,1.28642645648559E-16));
#120534=DIRECTION('ref_axis',(-0.406736643075801,-0.9135454576426,-7.47472011570615E-33));
#120535=DIRECTION('center_axis',(0.913545457642598,-0.406736643075807,0.));
#120536=DIRECTION('ref_axis',(0.406736643075807,0.913545457642598,0.));
#120537=DIRECTION('center_axis',(-1.21742612413517E-17,-5.72753959967198E-17,
-1.));
#120538=DIRECTION('ref_axis',(0.,1.,-1.12832121675104E-16));
#120539=DIRECTION('center_axis',(-0.406515100163544,-0.913644062717546,
0.));
#120540=DIRECTION('ref_axis',(0.913644062717546,-0.406515100163544,0.));
#120541=DIRECTION('center_axis',(0.48411028140672,-0.215539784135064,-0.848044713969326));
#120542=DIRECTION('ref_axis',(-0.868457761888285,1.62534225110956E-15,-0.495763165045559));
#120543=DIRECTION('center_axis',(0.484109806651295,-0.21553957276033,0.848045038708641));
#120544=DIRECTION('ref_axis',(0.868458052949953,2.8886639606392E-15,-0.495762655175212));
#120545=DIRECTION('center_axis',(0.484110321455164,-0.215539774370365,-0.848044693589288));
#120546=DIRECTION('ref_axis',(-0.772875576449771,0.349068641848483,-0.529919264233232));
#120547=DIRECTION('center_axis',(0.484110341087615,-0.215539810706674,-0.848044673146742));
#120548=DIRECTION('ref_axis',(-0.868457725299268,3.55645384105659E-15,-0.495763229140706));
#120549=DIRECTION('center_axis',(-0.484109823426766,0.21553960397576,-0.848045021198567));
#120550=DIRECTION('ref_axis',(0.776473315751262,-0.340990855186454,-0.529919264233196));
#120551=DIRECTION('center_axis',(0.484109857923801,-0.21553959558832,0.848045003637555));
#120552=DIRECTION('ref_axis',(0.868458021515976,-2.41205393455667E-15,-0.495762710240047));
#120553=DIRECTION('center_axis',(-0.406972488803041,-0.913440415876952,
0.));
#120554=DIRECTION('ref_axis',(0.913440415876952,-0.406972488803041,0.));
#120555=DIRECTION('center_axis',(0.913545457642598,-0.406736643075807,0.));
#120556=DIRECTION('ref_axis',(0.406736643075807,0.913545457642598,0.));
#120557=DIRECTION('center_axis',(-1.21742612413517E-17,-5.72753959967198E-17,
-1.));
#120558=DIRECTION('ref_axis',(0.,1.,0.));
#120559=DIRECTION('center_axis',(-0.406500770236728,-0.913650438514067,
2.49595411736509E-14));
#120560=DIRECTION('ref_axis',(0.913650438514067,-0.406500770236727,-1.61030417725217E-28));
#120561=DIRECTION('center_axis',(0.913545457642601,-0.406736643075801,-1.28642645648559E-16));
#120562=DIRECTION('ref_axis',(0.406736643075801,0.913545457642601,7.9109897830696E-31));
#120563=DIRECTION('center_axis',(0.791134794601138,-0.352268789800911,-0.500012436348953));
#120564=DIRECTION('ref_axis',(0.457186437804586,-0.202469153665354,0.8660177844026));
#120565=DIRECTION('center_axis',(-0.484110341087606,0.215539810706706,0.848044673146739));
#120566=DIRECTION('ref_axis',(0.868457725299272,-5.00491300951417E-15,0.495763229140701));
#120567=DIRECTION('center_axis',(-0.456777309432038,0.203370349885425,0.86602251147156));
#120568=DIRECTION('ref_axis',(-0.792963725161865,0.348150155216779,-0.499999999999951));
#120569=DIRECTION('center_axis',(0.456777317573163,-0.203370364581863,-0.866022503726379));
#120570=DIRECTION('ref_axis',(-0.88450703638216,-1.63558781625489E-15,-0.466526850878326));
#120571=DIRECTION('center_axis',(-0.484110321307456,0.215539774224879,0.848044693710585));
#120572=DIRECTION('ref_axis',(-0.776563258031751,0.340785973404991,-0.529919264233265));
#120573=DIRECTION('center_axis',(-0.484110281406723,0.215539784135065,0.848044713969325));
#120574=DIRECTION('ref_axis',(0.868457761888284,-9.9277303974391E-16,0.495763165045561));
#120575=DIRECTION('center_axis',(0.913545457642598,-0.406736643075807,0.));
#120576=DIRECTION('ref_axis',(0.406736643075807,0.913545457642598,0.));
#120577=DIRECTION('center_axis',(-0.913545457642598,0.406736643075807,0.));
#120578=DIRECTION('ref_axis',(-0.406736643075807,-0.913545457642598,0.));
#120579=DIRECTION('center_axis',(0.913545457642601,-0.406736643075801,-1.28642645648559E-16));
#120580=DIRECTION('ref_axis',(0.406736643075801,0.913545457642601,7.9109897830696E-31));
#120581=DIRECTION('center_axis',(0.913545457642598,-0.406736643075807,2.22228536467272E-14));
#120582=DIRECTION('ref_axis',(0.406736643075807,0.913545457642598,3.85652098937002E-31));
#120583=DIRECTION('center_axis',(0.913545457642601,-0.406736643075801,-1.28642645648559E-16));
#120584=DIRECTION('ref_axis',(0.406736643075801,0.913545457642601,7.9109897830696E-31));
#120585=DIRECTION('center_axis',(-0.791150459692759,0.352280597670772,-0.499979330205419));
#120586=DIRECTION('ref_axis',(0.456361522793348,-0.204240445643174,-0.866036951219296));
#120587=DIRECTION('center_axis',(0.456777441376069,-0.203370419702468,0.866022425483298));
#120588=DIRECTION('ref_axis',(0.884506966812062,6.03592299906791E-15,-0.466526982779053));
#120589=DIRECTION('center_axis',(0.456777449576405,-0.203370423353496,0.866022420300707));
#120590=DIRECTION('ref_axis',(-0.406736643068955,-0.913545457645649,-4.33598912519089E-12));
#120591=DIRECTION('center_axis',(-0.433017044461004,0.250002507183264,0.866022508719224));
#120592=DIRECTION('ref_axis',(0.499999999999256,0.866025403784868,-4.89547161594789E-13));
#120593=DIRECTION('center_axis',(-0.750008802378745,0.4329830941858,0.500012436349029));
#120594=DIRECTION('ref_axis',(0.432528431855697,-0.250863215188869,0.866017784402581));
#120595=DIRECTION('center_axis',(0.433017051950287,-0.250002511507195,-0.866022503726305));
#120596=DIRECTION('ref_axis',(-0.894424794863779,-2.9162281599034E-15,-0.447218387740136));
#120597=DIRECTION('center_axis',(0.86602540378444,-0.499999999999998,-6.09762352041363E-14));
#120598=DIRECTION('ref_axis',(0.499999999999998,0.86602540378444,8.28350179725319E-28));
#120599=DIRECTION('center_axis',(-0.866025403784438,0.500000000000001,1.2195101864901E-16));
#120600=DIRECTION('ref_axis',(-0.500000000000001,-0.866025403784438,6.92065314020432E-33));
#120601=DIRECTION('center_axis',(-0.866025403784433,0.50000000000001,0.));
#120602=DIRECTION('ref_axis',(-0.50000000000001,-0.866025403784433,0.));
#120603=DIRECTION('center_axis',(-0.866025403784438,0.500000000000001,1.2195101864901E-16));
#120604=DIRECTION('ref_axis',(-0.500000000000001,-0.866025403784438,6.92065314020432E-33));
#120605=DIRECTION('center_axis',(0.86602540378444,-0.499999999999998,0.));
#120606=DIRECTION('ref_axis',(0.499999999999998,0.86602540378444,0.));
#120607=DIRECTION('center_axis',(-0.458927830768609,0.264962106632866,-0.848045003637597));
#120608=DIRECTION('ref_axis',(-0.879478602053342,2.04159790904447E-15,0.475938429348062));
#120609=DIRECTION('center_axis',(0.433017169313211,-0.250002579266684,0.866022425483301));
#120610=DIRECTION('ref_axis',(0.894424730216421,1.52776146092203E-15,-0.447218517033097));
#120611=DIRECTION('center_axis',(0.458927795478264,-0.264962111234757,0.848045021297502));
#120612=DIRECTION('ref_axis',(0.7322669605685,-0.427750712277967,-0.529919264233206));
#120613=DIRECTION('center_axis',(-0.45892778216322,0.264962078570532,-0.848045038708636));
#120614=DIRECTION('ref_axis',(-0.879478631391242,-3.91934596708905E-15,
0.475938375135046));
#120615=DIRECTION('center_axis',(0.433017176052958,-0.250002595297057,0.866022417485747));
#120616=DIRECTION('ref_axis',(0.747715375894778,-0.436945896708641,-0.500000000000013));
#120617=DIRECTION('center_axis',(0.750027562856299,-0.432988827019191,0.499979330205145));
#120618=DIRECTION('ref_axis',(0.433476564275525,-0.249154705647712,-0.866036951219455));
#120619=DIRECTION('center_axis',(-0.500209992837911,-0.865904130412309,
0.));
#120620=DIRECTION('ref_axis',(0.865904130412309,-0.500209992837911,0.));
#120621=DIRECTION('center_axis',(-0.866025403784438,0.500000000000001,1.2195101864901E-16));
#120622=DIRECTION('ref_axis',(-0.500000000000001,-0.866025403784438,6.92065314020432E-33));
#120623=DIRECTION('center_axis',(0.866025403784433,-0.50000000000001,0.));
#120624=DIRECTION('ref_axis',(0.50000000000001,0.866025403784433,0.));
#120625=DIRECTION('center_axis',(-1.88658882409001E-17,-7.04084534449554E-17,
-1.));
#120626=DIRECTION('ref_axis',(0.,1.,-1.12832121675104E-16));
#120627=DIRECTION('center_axis',(-0.499789977759974,-0.86614662623062,0.));
#120628=DIRECTION('ref_axis',(0.86614662623062,-0.499789977759974,0.));
#120629=DIRECTION('center_axis',(0.458928232223209,-0.264962338412804,-0.848044713969316));
#120630=DIRECTION('ref_axis',(-0.879478359737741,-7.92594685885185E-17,
-0.475938877118704));
#120631=DIRECTION('center_axis',(0.458927782163206,-0.264962078570532,0.848045038708643));
#120632=DIRECTION('ref_axis',(0.879478631391249,-1.80847170028479E-16,-0.475938375135033));
#120633=DIRECTION('center_axis',(0.45892827307444,-0.264962332885194,-0.848044693589287));
#120634=DIRECTION('ref_axis',(-0.732154074464041,0.427943903613827,-0.529919264233207));
#120635=DIRECTION('center_axis',(0.458928288799672,-0.264962371077207,-0.848044673146733));
#120636=DIRECTION('ref_axis',(-0.879478325588501,4.31424957953392E-16,-0.475938940222427));
#120637=DIRECTION('center_axis',(-0.458927795586795,0.264962111363442,-0.848045021198564));
#120638=DIRECTION('ref_axis',(0.736576463604698,-0.420286434063858,-0.529919264233226));
#120639=DIRECTION('center_axis',(0.458927830768629,-0.264962106632886,0.848045003637581));
#120640=DIRECTION('ref_axis',(0.87947860205333,4.54286346810456E-15,-0.475938429348083));
#120641=DIRECTION('center_axis',(-0.500223573885338,-0.86589628485713,2.36549702850838E-14));
#120642=DIRECTION('ref_axis',(0.86589628485713,-0.500223573885338,2.17560721291705E-28));
#120643=DIRECTION('center_axis',(0.866025403784433,-0.50000000000001,0.));
#120644=DIRECTION('ref_axis',(0.50000000000001,0.866025403784433,0.));
#120645=DIRECTION('center_axis',(-1.88658882409001E-17,-7.04084534449554E-17,
-1.));
#120646=DIRECTION('ref_axis',(0.,1.,-1.20114286872534E-16));
#120647=DIRECTION('center_axis',(-0.499776392786186,-0.866154464985102,
-2.36620233737285E-14));
#120648=DIRECTION('ref_axis',(0.866154464985102,-0.499776392786186,2.10998669647211E-28));
#120649=DIRECTION('center_axis',(0.866025403784438,-0.500000000000001,-1.2195101864901E-16));
#120650=DIRECTION('ref_axis',(0.500000000000001,0.866025403784438,1.24416343873374E-30));
#120651=DIRECTION('center_axis',(0.749978760163569,-0.433035128829407,-0.500012436348552));
#120652=DIRECTION('ref_axis',(-0.433518133149823,0.249149002262184,-0.866017784402867));
#120653=DIRECTION('center_axis',(-0.458928288799668,0.264962371077193,0.84804467314674));
#120654=DIRECTION('ref_axis',(0.879478325588503,-1.89639858451521E-15,0.475938940222423));
#120655=DIRECTION('center_axis',(-0.433017045389765,0.250002496040436,0.866022511471538));
#120656=DIRECTION('ref_axis',(-0.752228186192807,0.429130231860971,-0.500000000000028));
#120657=DIRECTION('center_axis',(0.433017051950197,-0.250002511507151,-0.866022503726362));
#120658=DIRECTION('ref_axis',(-0.894424794863829,-5.98165056151269E-15,
-0.447218387740037));
#120659=DIRECTION('center_axis',(-0.458928272943999,0.264962332722854,0.848044693710598));
#120660=DIRECTION('ref_axis',(-0.736687329156677,0.420092076162478,-0.529919264233242));
#120661=DIRECTION('center_axis',(-0.458928232223181,0.264962338412833,0.848044713969322));
#120662=DIRECTION('ref_axis',(0.879478359737755,5.09289574828741E-15,0.475938877118678));
#120663=DIRECTION('center_axis',(0.866025403784433,-0.50000000000001,-1.36592399683214E-14));
#120664=DIRECTION('ref_axis',(0.50000000000001,0.866025403784433,-1.33215113601878E-31));
#120665=DIRECTION('center_axis',(-0.866025403784433,0.50000000000001,0.));
#120666=DIRECTION('ref_axis',(-0.50000000000001,-0.866025403784433,0.));
#120667=DIRECTION('center_axis',(0.866025403784438,-0.500000000000001,-1.2195101864901E-16));
#120668=DIRECTION('ref_axis',(0.500000000000001,0.866025403784438,1.24416343873374E-30));
#120669=DIRECTION('center_axis',(0.866025403784433,-0.50000000000001,0.));
#120670=DIRECTION('ref_axis',(0.50000000000001,0.866025403784433,0.));
#120671=DIRECTION('center_axis',(0.866025403784438,-0.500000000000001,-1.2195101864901E-16));
#120672=DIRECTION('ref_axis',(0.500000000000001,0.866025403784438,1.24416343873374E-30));
#120673=DIRECTION('center_axis',(-0.749993105181574,0.433048509462462,-0.4999793302052));
#120674=DIRECTION('ref_axis',(-0.432512586708856,0.250824363770665,0.866036951219436));
#120675=DIRECTION('center_axis',(0.433017169313192,-0.250002579266708,0.866022425483304));
#120676=DIRECTION('ref_axis',(0.894424730216429,-3.15083324732399E-15,-0.44721851703308));
#120677=DIRECTION('center_axis',(0.433017177087157,-0.250002583755012,0.866022420300588));
#120678=DIRECTION('ref_axis',(-0.499999999997495,-0.866025403785885,-1.67844740331651E-12));
#120679=DIRECTION('center_axis',(-0.404512553894058,0.293895573516091,0.866022508720042));
#120680=DIRECTION('ref_axis',(0.58778525229198,0.809016994375305,-3.49676543998341E-13));
#120681=DIRECTION('center_axis',(-0.700641118228541,0.509008435041967,0.500012436348926));
#120682=DIRECTION('ref_axis',(0.403936649474811,-0.294700492550331,0.866017784402639));
#120683=DIRECTION('center_axis',(0.404512560891457,-0.293895578600019,-0.866022503726315));
#120684=DIRECTION('ref_axis',(-0.906035256115487,-3.15407140147818E-15,
-0.423202214875754));
#120685=DIRECTION('center_axis',(0.809016994374931,-0.587785252292496,0.));
#120686=DIRECTION('ref_axis',(0.587785252292496,0.809016994374931,0.));
#120687=DIRECTION('center_axis',(-0.809016994374947,0.587785252292474,1.13923270769252E-16));
#120688=DIRECTION('ref_axis',(-0.587785252292474,-0.809016994374947,8.80720662300256E-33));
#120689=DIRECTION('center_axis',(-0.809016994374931,0.587785252292496,-3.21147992436134E-14));
#120690=DIRECTION('ref_axis',(-0.587785252292496,-0.809016994374931,2.25632648858384E-30));
#120691=DIRECTION('center_axis',(-0.809016994374947,0.587785252292474,1.13923270769252E-16));
#120692=DIRECTION('ref_axis',(-0.587785252292474,-0.809016994374947,8.80720662300256E-33));
#120693=DIRECTION('center_axis',(0.80901699437495,-0.58778525229247,0.));
#120694=DIRECTION('ref_axis',(0.58778525229247,0.80901699437495,0.));
#120695=DIRECTION('center_axis',(-0.428717694262756,0.311481637390311,-0.848045003637588));
#120696=DIRECTION('ref_axis',(-0.892442058026273,-6.51151864539323E-15,
0.451162025292277));
#120697=DIRECTION('center_axis',(0.404512670528671,-0.293895658256118,0.866022425483293));
#120698=DIRECTION('ref_axis',(0.906035197473499,1.81134782246753E-15,-0.423202340422589));
#120699=DIRECTION('center_axis',(0.428717658681014,-0.311481638283158,0.848045021297519));
#120700=DIRECTION('ref_axis',(0.683543400918347,-0.501950189217554,-0.529919264233186));
#120701=DIRECTION('center_axis',(-0.428717648856913,0.311481604401034,-0.848045038708652));
#120702=DIRECTION('ref_axis',(-0.89244208477774,-4.94272061273143E-15,0.451161972375288));
#120703=DIRECTION('center_axis',(0.404512675553166,-0.293895674906847,0.866022417485753));
#120704=DIRECTION('ref_axis',(0.69794602971643,-0.512709800572455,-0.500000000000025));
#120705=DIRECTION('center_axis',(0.700659176689928,-0.509016097474107,0.499979330205182));
#120706=DIRECTION('ref_axis',(0.405058175792842,-0.29310044924206,-0.866036951219449));
#120707=DIRECTION('center_axis',(-0.587981418248406,-0.808874435122407,
7.63199572093835E-14));
#120708=DIRECTION('ref_axis',(0.808874435122407,-0.587981418248406,4.48144986036732E-28));
#120709=DIRECTION('center_axis',(-0.809016994374947,0.587785252292474,1.13923270769252E-16));
#120710=DIRECTION('ref_axis',(-0.587785252292474,-0.809016994374947,8.80720662300256E-33));
#120711=DIRECTION('center_axis',(0.809016994374969,-0.587785252292444,0.));
#120712=DIRECTION('ref_axis',(0.587785252292444,0.809016994374969,0.));
#120713=DIRECTION('center_axis',(-2.68936361206584E-17,-8.27701011433319E-17,
-1.));
#120714=DIRECTION('ref_axis',(0.,1.,-1.12832121675104E-16));
#120715=DIRECTION('center_axis',(-0.587589051772239,-0.809159506053906,
0.));
#120716=DIRECTION('ref_axis',(0.809159506053906,-0.587589051772239,0.));
#120717=DIRECTION('center_axis',(0.428718069290544,-0.311481909863919,-0.848044713969325));
#120718=DIRECTION('ref_axis',(-0.892441837073393,5.69339720065885E-15,-0.451162462358149));
#120719=DIRECTION('center_axis',(0.428717648856975,-0.311481604401136,0.848045038708583));
#120720=DIRECTION('ref_axis',(0.892442084777698,-4.42555422208939E-15,-0.451161972375372));
#120721=DIRECTION('center_axis',(0.428718110495911,-0.311481908636537,-0.848044693589292));
#120722=DIRECTION('ref_axis',(-0.683410939222547,0.502130522419756,-0.529919264233165));
#120723=DIRECTION('center_axis',(0.428718122142701,-0.311481948263287,-0.848044673146729));
#120724=DIRECTION('ref_axis',(-0.892441805934776,-6.12251068898412E-15,
-0.45116252395326));
#120725=DIRECTION('center_axis',(-0.428717658775709,0.311481638422204,-0.848045021198577));
#120726=DIRECTION('ref_axis',(0.688609525574901,-0.494977266833597,-0.529919264233195));
#120727=DIRECTION('center_axis',(0.428717694262811,-0.31148163739035,0.848045003637546));
#120728=DIRECTION('ref_axis',(0.892442058026239,-8.51765461603545E-15,-0.451162025292345));
#120729=DIRECTION('center_axis',(-0.587994104813606,-0.808865212939984,
0.));
#120730=DIRECTION('ref_axis',(0.808865212939984,-0.587994104813606,0.));
#120731=DIRECTION('center_axis',(0.809016994374931,-0.587785252292496,-7.63170283020858E-14));
#120732=DIRECTION('ref_axis',(0.587785252292496,0.809016994374931,-5.02862541378261E-30));
#120733=DIRECTION('center_axis',(-2.68936361206584E-17,-8.27701011433319E-17,
-1.));
#120734=DIRECTION('ref_axis',(0.,1.,-1.20114286872534E-16));
#120735=DIRECTION('center_axis',(-0.587576360591353,-0.80916872188328,-3.21033860361202E-14));
#120736=DIRECTION('ref_axis',(0.80916872188328,-0.587576360591353,4.80687827587565E-28));
#120737=DIRECTION('center_axis',(0.809016994374947,-0.587785252292474,-1.13923270769252E-16));
#120738=DIRECTION('ref_axis',(0.587785252292474,0.809016994374947,1.19410145339382E-30));
#120739=DIRECTION('center_axis',(0.700605801486325,-0.509057044367352,-0.500012436349018));
#120740=DIRECTION('ref_axis',(-0.40510011313772,0.293099122199729,-0.866017784402581));
#120741=DIRECTION('center_axis',(-0.428718122142726,0.311481948263255,0.848044673146729));
#120742=DIRECTION('ref_axis',(0.892441805934764,-1.37149456183714E-15,0.451162523953283));
#120743=DIRECTION('center_axis',(-0.404512555984775,0.293895562530571,0.866022511471558));
#120744=DIRECTION('ref_axis',(-0.703251077802595,0.505408667881258,-0.49999999999998));
#120745=DIRECTION('center_axis',(0.404512560891371,-0.293895578599957,-0.866022503726376));
#120746=DIRECTION('ref_axis',(-0.906035256115534,-6.84927325568381E-15,
-0.423202214875654));
#120747=DIRECTION('center_axis',(-0.428718110383012,0.311481908461646,0.848044693710603));
#120748=DIRECTION('ref_axis',(-0.688740099725524,0.494795562252288,-0.529919264233258));
#120749=DIRECTION('center_axis',(-0.428718069290536,0.311481909863913,0.848044713969331));
#120750=DIRECTION('ref_axis',(0.892441837073398,-1.59472440562988E-15,0.451162462358138));
#120751=DIRECTION('center_axis',(0.809016994374931,-0.587785252292496,0.));
#120752=DIRECTION('ref_axis',(0.587785252292496,0.809016994374931,0.));
#120753=DIRECTION('center_axis',(-0.80901699437495,0.58778525229247,0.));
#120754=DIRECTION('ref_axis',(-0.58778525229247,-0.80901699437495,0.));
#120755=DIRECTION('center_axis',(0.809016994374947,-0.587785252292474,-1.13923270769252E-16));
#120756=DIRECTION('ref_axis',(0.587785252292474,0.809016994374947,1.19410145339382E-30));
#120757=DIRECTION('center_axis',(0.809016994374931,-0.587785252292496,-4.42022290584682E-14));
#120758=DIRECTION('ref_axis',(0.587785252292496,0.809016994374931,4.35974171970421E-30));
#120759=DIRECTION('center_axis',(0.809016994374947,-0.587785252292474,-1.13923270769252E-16));
#120760=DIRECTION('ref_axis',(0.587785252292474,0.809016994374947,1.19410145339382E-30));
#120761=DIRECTION('center_axis',(-0.700618669263857,0.509071851162881,-0.4999793302053));
#120762=DIRECTION('ref_axis',(-0.403924952204904,0.29466019770054,0.866036951219372));
#120763=DIRECTION('center_axis',(0.404512670528677,-0.293895658256122,0.866022425483289));
#120764=DIRECTION('ref_axis',(0.906035197473497,3.93346248258234E-15,-0.423202340422595));
#120765=DIRECTION('center_axis',(0.404512677786642,-0.293895663529335,0.866022420303616));
#120766=DIRECTION('ref_axis',(-0.58778525229999,-0.809016994369486,5.3500510981539E-12));
#120767=DIRECTION('center_axis',(-0.371576139133635,0.334568658440529,0.866022508723559));
#120768=DIRECTION('ref_axis',(0.669130606356872,0.743144825479183,-1.53857679357235E-12));
#120769=DIRECTION('center_axis',(-0.643597063369161,0.57945697296553,0.500012436349555));
#120770=DIRECTION('ref_axis',(0.370919252615107,-0.33530896966599,0.86601778440225));
#120771=DIRECTION('center_axis',(0.371576145565852,-0.334568664232084,-0.866022503726309));
#120772=DIRECTION('ref_axis',(-0.918982183096513,-7.2095623261364E-15,-0.394299058014557));
#120773=DIRECTION('center_axis',(0.743144825477406,-0.669130606358845,-7.71624360992626E-14));
#120774=DIRECTION('ref_axis',(0.669130606358845,0.743144825477406,4.74868592476285E-30));
#120775=DIRECTION('center_axis',(-0.743144825477393,0.669130606358859,1.04647355694969E-16));
#120776=DIRECTION('ref_axis',(-0.669130606358859,-0.743144825477393,1.70053300922835E-32));
#120777=DIRECTION('center_axis',(-0.743144825477406,0.669130606358845,0.));
#120778=DIRECTION('ref_axis',(-0.669130606358845,-0.743144825477406,0.));
#120779=DIRECTION('center_axis',(-0.743144825477393,0.669130606358859,1.04647355694969E-16));
#120780=DIRECTION('ref_axis',(-0.669130606358859,-0.743144825477393,1.70053300922835E-32));
#120781=DIRECTION('center_axis',(0.743144825477382,-0.669130606358872,0.));
#120782=DIRECTION('ref_axis',(0.669130606358872,0.743144825477382,0.));
#120783=DIRECTION('center_axis',(-0.393810436983632,0.354588510146749,-0.848045003637584));
#120784=DIRECTION('ref_axis',(-0.906978223357768,-5.83873457091855E-16,
0.421177518814558));
#120785=DIRECTION('center_axis',(0.371576246276125,-0.334568754912021,0.866022425483293));
#120786=DIRECTION('ref_axis',(0.918982131463643,6.34168247799913E-15,-0.394299178353873));
#120787=DIRECTION('center_axis',(0.393810401508524,-0.354588507309826,0.848045021297504));
#120788=DIRECTION('ref_axis',(0.627330796737913,-0.570650194829292,-0.52991926423321));
#120789=DIRECTION('center_axis',(-0.393810395274862,0.354588472592004,-0.848045038708633));
#120790=DIRECTION('ref_axis',(-0.906978247051285,1.62635303421704E-15,0.421177467792116));
#120791=DIRECTION('center_axis',(0.37157624953938,-0.334568771989208,0.866022417485761));
#120792=DIRECTION('ref_axis',(0.640529840782192,-0.582856348569324,-0.499999999999975));
#120793=DIRECTION('center_axis',(0.643614221961268,-0.579466481046713,0.499979330205291));
#120794=DIRECTION('ref_axis',(0.372201885200888,-0.333834922941829,-0.866036951219362));
#120795=DIRECTION('center_axis',(-0.669310796197597,-0.742982542253409,
0.));
#120796=DIRECTION('ref_axis',(0.742982542253409,-0.669310796197597,0.));
#120797=DIRECTION('center_axis',(-0.743144825477393,0.669130606358859,1.04647355694969E-16));
#120798=DIRECTION('ref_axis',(-0.669130606358859,-0.743144825477393,1.70053300922835E-32));
#120799=DIRECTION('center_axis',(0.743144825477382,-0.669130606358872,0.));
#120800=DIRECTION('ref_axis',(0.669130606358872,0.743144825477382,0.));
#120801=DIRECTION('center_axis',(-3.61695511949416E-17,-9.42249022928248E-17,
-1.));
#120802=DIRECTION('ref_axis',(0.,1.,-1.12832121675104E-16));
#120803=DIRECTION('center_axis',(-0.668950377172406,-0.743307065001333,
0.));
#120804=DIRECTION('ref_axis',(0.743307065001333,-0.668950377172406,0.));
#120805=DIRECTION('center_axis',(0.393810781475684,-0.35458882032882,-0.848044713969332));
#120806=DIRECTION('ref_axis',(-0.906978027661852,2.89845252510014E-15,-0.421177940232649));
#120807=DIRECTION('center_axis',(0.39381039527486,-0.354588472592002,0.848045038708635));
#120808=DIRECTION('ref_axis',(0.906978247051286,-2.65749036098971E-15,-0.421177467792113));
#120809=DIRECTION('center_axis',(0.393810822586016,-0.354588823412691,-0.848044693589276));
#120810=DIRECTION('ref_axis',(-0.627180210717368,0.570815694142259,-0.529919264233156));
#120811=DIRECTION('center_axis',(0.393810830024562,-0.354588864042303,-0.848044673146736));
#120812=DIRECTION('ref_axis',(-0.906978000082633,-7.8483346287888E-15,-0.421177999622614));
#120813=DIRECTION('center_axis',(-0.393810401582675,0.354588507464094,-0.848045021198567));
#120814=DIRECTION('ref_axis',(0.633098037491572,-0.564245025072303,-0.529919264233219));
#120815=DIRECTION('center_axis',(0.393810436983644,-0.35458851014676,0.848045003637574));
#120816=DIRECTION('ref_axis',(0.90697822335776,-1.35612861251301E-15,-0.421177518814574));
#120817=DIRECTION('center_axis',(-0.6693224492839,-0.74297204448391,3.65697438038149E-14));
#120818=DIRECTION('ref_axis',(0.74297204448391,-0.6693224492839,5.21231353425566E-29));
#120819=DIRECTION('center_axis',(0.743144825477406,-0.669130606358845,3.65592620896166E-14));
#120820=DIRECTION('ref_axis',(0.669130606358845,0.743144825477406,-1.6162287319392E-30));
#120821=DIRECTION('center_axis',(-3.61695511949416E-17,-9.42249022928248E-17,
-1.));
#120822=DIRECTION('ref_axis',(0.,1.,-1.20114286872534E-16));
#120823=DIRECTION('center_axis',(-0.668938718831589,-0.743317556935091,
0.));
#120824=DIRECTION('ref_axis',(0.743317556935091,-0.668938718831589,0.));
#120825=DIRECTION('center_axis',(0.743144825477393,-0.669130606358859,-1.04647355694969E-16));
#120826=DIRECTION('ref_axis',(0.669130606358859,0.743144825477393,-1.0963218983187E-31));
#120827=DIRECTION('center_axis',(0.643556859035248,-0.579501624401408,-0.500012436350153));
#120828=DIRECTION('ref_axis',(-0.372243731481368,0.333837986862428,-0.866017784401954));
#120829=DIRECTION('center_axis',(-0.393810830024468,0.354588864042396,0.848044673146741));
#120830=DIRECTION('ref_axis',(0.90697800008267,-6.46020788503429E-15,0.421177999622535));
#120831=DIRECTION('center_axis',(-0.371576142362482,0.33456864774147,0.866022511471533));
#120832=DIRECTION('ref_axis',(-0.646569003441366,0.576149740769561,-0.500000000000006));
#120833=DIRECTION('center_axis',(0.371576145565767,-0.334568664232008,-0.866022503726374));
#120834=DIRECTION('ref_axis',(-0.918982183096555,4.84816140359523E-15,-0.39429905801446));
#120835=DIRECTION('center_axis',(-0.3938108224892,0.354588823230052,0.848044693710601));
#120836=DIRECTION('ref_axis',(-0.633246889647289,0.564077964599343,-0.529919264233238));
#120837=DIRECTION('center_axis',(-0.393810781475669,0.354588820328864,0.848044713969321));
#120838=DIRECTION('ref_axis',(0.906978027661855,-6.11429089785958E-15,0.421177940232642));
#120839=DIRECTION('center_axis',(0.743144825477406,-0.669130606358845,3.65592620896146E-14));
#120840=DIRECTION('ref_axis',(0.669130606358845,0.743144825477406,1.03271697859918E-30));
#120841=DIRECTION('center_axis',(-0.743144825477406,0.669130606358845,0.));
#120842=DIRECTION('ref_axis',(-0.669130606358845,-0.743144825477406,0.));
#120843=DIRECTION('center_axis',(0.743144825477393,-0.669130606358859,-1.04647355694969E-16));
#120844=DIRECTION('ref_axis',(0.669130606358859,0.743144825477393,-1.0963218983187E-31));
#120845=DIRECTION('center_axis',(0.743144825477406,-0.669130606358845,4.06031740096457E-14));
#120846=DIRECTION('ref_axis',(0.669130606358845,0.743144825477406,2.80523855531594E-30));
#120847=DIRECTION('center_axis',(0.743144825477393,-0.669130606358859,-1.04647355694969E-16));
#120848=DIRECTION('ref_axis',(0.669130606358859,0.743144825477393,-1.0963218983187E-31));
#120849=DIRECTION('center_axis',(-0.643568108591829,0.579517695132094,-0.499979330205082));
#120850=DIRECTION('ref_axis',(-0.3709118314048,0.335267672832272,0.866036951219502));
#120851=DIRECTION('center_axis',(0.371576246276117,-0.334568754912014,0.866022425483298));
#120852=DIRECTION('ref_axis',(0.918982131463646,3.28768502367003E-15,-0.394299178353865));
#120853=DIRECTION('center_axis',(0.371576252946115,-0.334568760917775,0.86602242030127));
#120854=DIRECTION('ref_axis',(-0.66913060635473,-0.743144825481112,-3.25199184387666E-12));
#120855=DIRECTION('center_axis',(-0.334568658443921,0.371576139137501,0.86602250872059));
#120856=DIRECTION('ref_axis',(0.743144825478317,0.669130606357834,7.34320742387398E-13));
#120857=DIRECTION('center_axis',(-0.579501624400846,0.643556859036295,0.500012436349456));
#120858=DIRECTION('ref_axis',(0.333837986833296,-0.372243731506635,0.866017784402323));
#120859=DIRECTION('center_axis',(0.334568664232049,-0.371576145565884,-0.866022503726308));
#120860=DIRECTION('ref_axis',(1.54577326889484E-15,0.9189821830965,-0.394299058014588));
#120861=DIRECTION('center_axis',(0.669130606358845,-0.743144825477406,0.));
#120862=DIRECTION('ref_axis',(0.743144825477406,0.669130606358845,0.));
#120863=DIRECTION('center_axis',(-0.669130606358857,0.743144825477395,9.42249022928245E-17));
#120864=DIRECTION('ref_axis',(-0.743144825477395,-0.669130606358857,-2.92763886583203E-33));
#120865=DIRECTION('center_axis',(-0.669130606358845,0.743144825477406,0.));
#120866=DIRECTION('ref_axis',(-0.743144825477406,-0.669130606358845,0.));
#120867=DIRECTION('center_axis',(-0.669130606358857,0.743144825477395,9.42249022928245E-17));
#120868=DIRECTION('ref_axis',(-0.743144825477395,-0.669130606358857,-2.92763886583203E-33));
#120869=DIRECTION('center_axis',(0.669130606358872,-0.743144825477382,0.));
#120870=DIRECTION('ref_axis',(0.743144825477382,0.669130606358872,0.));
#120871=DIRECTION('center_axis',(-0.354588510146771,0.393810436983657,-0.848045003637563));
#120872=DIRECTION('ref_axis',(4.10739333192291E-15,0.906978223357754,0.421177518814587));
#120873=DIRECTION('center_axis',(0.334568754912014,-0.371576246276117,0.866022425483298));
#120874=DIRECTION('ref_axis',(-3.2863782672971E-15,-0.918982131463647,-0.394299178353865));
#120875=DIRECTION('center_axis',(0.354588475166891,-0.393810430450173,0.848045021297495));
#120876=DIRECTION('ref_axis',(0.564245025068685,-0.633098037494793,-0.529919264233223));
#120877=DIRECTION('center_axis',(-0.354588472592013,0.393810395274872,-0.848045038708624));
#120878=DIRECTION('ref_axis',(2.79096370469408E-15,0.90697824705128,0.421177467792126));
#120879=DIRECTION('center_axis',(0.334568756368268,-0.371576263604501,0.866022417485777));
#120880=DIRECTION('ref_axis',(0.57609587287032,-0.646617000442945,-0.499999999999953));
#120881=DIRECTION('center_axis',(0.579517695132538,-0.643568108591555,0.499979330204919));
#120882=DIRECTION('ref_axis',(0.335267672837596,-0.370911831399782,-0.86603695121959));
#120883=DIRECTION('center_axis',(-0.743307065001336,-0.668950377172403,
0.));
#120884=DIRECTION('ref_axis',(0.668950377172402,-0.743307065001336,0.));
#120885=DIRECTION('center_axis',(-0.669130606358857,0.743144825477395,9.42249022928245E-17));
#120886=DIRECTION('ref_axis',(-0.743144825477395,-0.669130606358857,-2.92763886583203E-33));
#120887=DIRECTION('center_axis',(0.669130606358872,-0.743144825477382,0.));
#120888=DIRECTION('ref_axis',(0.743144825477382,0.669130606358872,0.));
#120889=DIRECTION('center_axis',(-4.6592004597086E-17,-1.04647355694969E-16,
-1.));
#120890=DIRECTION('ref_axis',(0.,1.,-1.12832121675104E-16));
#120891=DIRECTION('center_axis',(-0.742982542253406,-0.669310796197601,
0.));
#120892=DIRECTION('ref_axis',(0.669310796197601,-0.742982542253406,0.));
#120893=DIRECTION('center_axis',(0.354588820328813,-0.393810781475714,-0.848044713969321));
#120894=DIRECTION('ref_axis',(8.39746514209146E-15,0.906978027661839,-0.421177940232676));
#120895=DIRECTION('center_axis',(0.354588472591992,-0.393810395274849,0.848045038708644));
#120896=DIRECTION('ref_axis',(7.73991416207292E-15,-0.906978247051291,-0.421177467792101));
#120897=DIRECTION('center_axis',(0.354588860891521,-0.393810788839952,-0.848044693589264));
#120898=DIRECTION('ref_axis',(-0.564077964590164,0.633246889655487,-0.529919264233212));
#120899=DIRECTION('center_axis',(0.354588864042362,-0.393810830024499,-0.848044673146741));
#120900=DIRECTION('ref_axis',(3.45335519356911E-15,0.906978000082659,-0.421177999622559));
#120901=DIRECTION('center_axis',(-0.354588475218221,0.393810430617001,-0.848045021198562));
#120902=DIRECTION('ref_axis',(0.570650194826636,-0.627330796740326,-0.529919264233213));
#120903=DIRECTION('center_axis',(0.35458851014676,-0.393810436983644,0.848045003637574));
#120904=DIRECTION('ref_axis',(1.6043859838781E-15,-0.906978223357761,-0.421177518814573));
#120905=DIRECTION('center_axis',(-0.743317556935091,-0.668938718831589,
0.));
#120906=DIRECTION('ref_axis',(0.668938718831589,-0.743317556935091,0.));
#120907=DIRECTION('center_axis',(0.669130606358845,-0.743144825477406,0.));
#120908=DIRECTION('ref_axis',(0.743144825477406,0.669130606358845,0.));
#120909=DIRECTION('center_axis',(-4.6592004597086E-17,-1.04647355694969E-16,
-1.));
#120910=DIRECTION('ref_axis',(0.,1.,-1.20114286872534E-16));
#120911=DIRECTION('center_axis',(-0.742972044483927,-0.669322449283882,
4.02398997762828E-15));
#120912=DIRECTION('ref_axis',(0.669322449283881,-0.742972044483927,-6.6843319428275E-29));
#120913=DIRECTION('center_axis',(0.669130606358857,-0.743144825477395,-9.42249022928245E-17));
#120914=DIRECTION('ref_axis',(0.743144825477395,0.669130606358857,1.50824901715581E-30));
#120915=DIRECTION('center_axis',(0.579456972966088,-0.643597063368669,-0.500012436349541));
#120916=DIRECTION('ref_axis',(-0.335308969655252,0.370919252624765,-0.866017784402271));
#120917=DIRECTION('center_axis',(-0.354588864042302,0.393810830024563,0.848044673146736));
#120918=DIRECTION('ref_axis',(-8.30756835896895E-15,-0.906978000082633,
0.421177999622615));
#120919=DIRECTION('center_axis',(-0.334568662772257,0.371576128828625,0.866022511471565));
#120920=DIRECTION('ref_axis',(-0.582802983772218,0.640578396534151,-0.499999999999936));
#120921=DIRECTION('center_axis',(0.334568664232006,-0.371576145565766,-0.866022503726375));
#120922=DIRECTION('ref_axis',(-5.31150746435353E-15,0.918982183096555,-0.394299058014458));
#120923=DIRECTION('center_axis',(-0.354588860817823,0.393810788644961,0.848044693710628));
#120924=DIRECTION('ref_axis',(-0.570815694139697,0.627180210719711,-0.529919264233142));
#120925=DIRECTION('center_axis',(-0.354588820328737,0.39381078147576,0.848044713969332));
#120926=DIRECTION('ref_axis',(2.72603440059969E-15,-0.906978027661821,0.421177940232716));
#120927=DIRECTION('center_axis',(0.669130606358845,-0.743144825477406,-4.04391192003352E-15));
#120928=DIRECTION('ref_axis',(0.743144825477406,0.669130606358845,-2.84816967279441E-31));
#120929=DIRECTION('center_axis',(-0.669130606358875,0.743144825477379,0.));
#120930=DIRECTION('ref_axis',(-0.743144825477379,-0.669130606358875,0.));
#120931=DIRECTION('center_axis',(0.669130606358857,-0.743144825477395,-9.42249022928245E-17));
#120932=DIRECTION('ref_axis',(0.743144825477395,0.669130606358857,1.50824901715581E-30));
#120933=DIRECTION('center_axis',(0.669130606358845,-0.743144825477406,0.));
#120934=DIRECTION('ref_axis',(0.743144825477406,0.669130606358845,0.));
#120935=DIRECTION('center_axis',(0.669130606358857,-0.743144825477395,-9.42249022928245E-17));
#120936=DIRECTION('ref_axis',(0.743144825477395,0.669130606358857,1.50824901715581E-30));
#120937=DIRECTION('center_axis',(-0.579466481046794,0.643614221961154,-0.499979330205343));
#120938=DIRECTION('ref_axis',(-0.333834922953757,0.372201885190229,0.866036951219345));
#120939=DIRECTION('center_axis',(0.334568754912021,-0.371576246276125,0.866022425483293));
#120940=DIRECTION('ref_axis',(-6.32948812453082E-15,-0.918982131463643,
-0.394299178353873));
#120941=DIRECTION('center_axis',(0.334568760919757,-0.371576252948344,0.866022420299548));
#120942=DIRECTION('ref_axis',(-0.743144825478174,-0.669130606357993,6.99353084714793E-13));
#120943=DIRECTION('center_axis',(-0.293895573513778,0.404512553890826,0.866022508722336));
#120944=DIRECTION('ref_axis',(0.80901699437535,0.587785252291919,4.19611852796817E-13));
#120945=DIRECTION('center_axis',(-0.509057044367578,0.700605801486098,0.500012436349106));
#120946=DIRECTION('ref_axis',(0.293099122201432,-0.405100113136594,0.866017784402531));
#120947=DIRECTION('center_axis',(0.293895578600017,-0.40451256089147,-0.86602250372631));
#120948=DIRECTION('ref_axis',(6.99855896983189E-15,0.906035256115482,-0.423202214875765));
#120949=DIRECTION('center_axis',(0.587785252292434,-0.809016994374976,0.));
#120950=DIRECTION('ref_axis',(0.809016994374976,0.587785252292434,0.));
#120951=DIRECTION('center_axis',(-0.587785252292471,0.809016994374949,8.27701011433315E-17));
#120952=DIRECTION('ref_axis',(-0.809016994374949,-0.587785252292471,1.88536659549102E-32));
#120953=DIRECTION('center_axis',(-0.587785252292496,0.809016994374931,0.));
#120954=DIRECTION('ref_axis',(-0.809016994374931,-0.587785252292496,0.));
#120955=DIRECTION('center_axis',(-0.587785252292471,0.809016994374949,8.27701011433315E-17));
#120956=DIRECTION('ref_axis',(-0.809016994374949,-0.587785252292471,1.54176213488025E-33));
#120957=DIRECTION('center_axis',(0.58778525229247,-0.80901699437495,0.));
#120958=DIRECTION('ref_axis',(0.80901699437495,0.58778525229247,0.));
#120959=DIRECTION('center_axis',(-0.311481637390324,0.428717694262775,-0.848045003637574));
#120960=DIRECTION('ref_axis',(-8.00971604565638E-16,0.892442058026262,0.451162025292301));
#120961=DIRECTION('center_axis',(0.293895658256083,-0.404512670528688,0.866022425483297));
#120962=DIRECTION('ref_axis',(8.0628843439915E-15,-0.906035197473492,-0.423202340422605));
#120963=DIRECTION('center_axis',(0.311481603279599,-0.428717684112632,0.848045021297497));
#120964=DIRECTION('ref_axis',(0.494977266813993,-0.688609525588986,-0.529919264233205));
#120965=DIRECTION('center_axis',(-0.31148160440103,0.428717648856906,-0.848045038708657));
#120966=DIRECTION('ref_axis',(2.39813197791476E-15,0.892442084777744,0.451161972375281));
#120967=DIRECTION('center_axis',(0.293895657890439,-0.404512687916314,0.866022417485751));
#120968=DIRECTION('ref_axis',(0.505350078027568,-0.703293181139626,-0.500000000000036));
#120969=DIRECTION('center_axis',(0.509071851162742,-0.700618669263935,0.499979330205332));
#120970=DIRECTION('ref_axis',(0.294660197708544,-0.403924952199123,-0.866036951219345));
#120971=DIRECTION('center_axis',(-0.809159506053914,-0.587589051772227,
0.));
#120972=DIRECTION('ref_axis',(0.587589051772227,-0.809159506053914,0.));
#120973=DIRECTION('center_axis',(-0.587785252292471,0.809016994374949,8.27701011433315E-17));
#120974=DIRECTION('ref_axis',(-0.809016994374949,-0.587785252292471,1.88536659549102E-32));
#120975=DIRECTION('center_axis',(0.58778525229246,-0.809016994374957,0.));
#120976=DIRECTION('ref_axis',(0.809016994374957,0.58778525229246,0.));
#120977=DIRECTION('center_axis',(-5.8046805746579E-17,-1.13923270769252E-16,
-1.));
#120978=DIRECTION('ref_axis',(0.,1.,-1.12832121675104E-16));
#120979=DIRECTION('center_axis',(-0.808874435122371,-0.587981418248456,
0.));
#120980=DIRECTION('ref_axis',(0.587981418248456,-0.808874435122371,0.));
#120981=DIRECTION('center_axis',(0.311481909863959,-0.42871806929052,-0.848044713969322));
#120982=DIRECTION('ref_axis',(-4.58604169299522E-15,0.892441837073402,-0.45116246235813));
#120983=DIRECTION('center_axis',(0.311481604401026,-0.428717648856901,0.848045038708661));
#120984=DIRECTION('ref_axis',(-4.08016432328408E-16,-0.892442084777747,
-0.451161972375276));
#120985=DIRECTION('center_axis',(0.311481949429352,-0.428718080858207,-0.848044693589286));
#120986=DIRECTION('ref_axis',(-0.49479556222845,0.688740099742701,-0.529919264233191));
#120987=DIRECTION('center_axis',(0.311481948263326,-0.428718122142675,-0.848044673146728));
#120988=DIRECTION('ref_axis',(-9.98849586125472E-16,0.892441805934786,-0.451162523953241));
#120989=DIRECTION('center_axis',(-0.311481603317813,0.428717684280574,-0.848045021198561));
#120990=DIRECTION('ref_axis',(0.501950189215672,-0.683543400919725,-0.529919264233192));
#120991=DIRECTION('center_axis',(0.311481637390342,-0.4287176942628,0.848045003637555));
#120992=DIRECTION('ref_axis',(-8.8971283331398E-15,-0.892442058026248,-0.451162025292327));
#120993=DIRECTION('center_axis',(-0.809168721883308,-0.587576360591314,
1.08417291060497E-13));
#120994=DIRECTION('ref_axis',(0.587576360591314,-0.809168721883308,-1.4872443511391E-27));
#120995=DIRECTION('center_axis',(0.587785252292496,-0.809016994374931,4.42022290584706E-14));
#120996=DIRECTION('ref_axis',(0.809016994374931,0.587785252292496,1.60275226051148E-30));
#120997=DIRECTION('center_axis',(-5.8046805746579E-17,-1.13923270769252E-16,
-1.));
#120998=DIRECTION('ref_axis',(0.,1.,-1.20114286872534E-16));
#120999=DIRECTION('center_axis',(-0.808865212939984,-0.587994104813606,
0.));
#121000=DIRECTION('ref_axis',(0.587994104813606,-0.808865212939984,0.));
#121001=DIRECTION('center_axis',(0.587785252292471,-0.809016994374949,-8.27701011433315E-17));
#121002=DIRECTION('ref_axis',(0.809016994374949,0.587785252292471,6.81387014938251E-31));
#121003=DIRECTION('center_axis',(0.509008435040905,-0.700641118228933,-0.500012436349457));
#121004=DIRECTION('ref_axis',(-0.294700492553427,0.403936649473218,-0.866017784402329));
#121005=DIRECTION('center_axis',(-0.311481948263287,0.428718122142701,0.848044673146729));
#121006=DIRECTION('ref_axis',(-6.11337967909926E-15,-0.892441805934776,
0.45116252395326));
#121007=DIRECTION('center_axis',(-0.293895578892578,0.40451254409714,0.86602251147153));
#121008=DIRECTION('ref_axis',(-0.512651652659763,0.697988741331279,-0.499999999999991));
#121009=DIRECTION('center_axis',(0.293895578599952,-0.404512560891364,-0.866022503726381));
#121010=DIRECTION('ref_axis',(4.4423106715044E-15,0.906035256115537,-0.423202214875647));
#121011=DIRECTION('center_axis',(-0.311481949376662,0.428718080656496,0.848044693710611));
#121012=DIRECTION('ref_axis',(-0.502130522402205,0.683410939235411,-0.529919264233206));
#121013=DIRECTION('center_axis',(-0.311481909863924,0.42871806929054,0.848044713969325));
#121014=DIRECTION('ref_axis',(-5.18787663535866E-16,-0.892441837073395,
0.451162462358144));
#121015=DIRECTION('center_axis',(0.587785252292496,-0.809016994374931,0.));
#121016=DIRECTION('ref_axis',(0.809016994374931,0.587785252292496,0.));
#121017=DIRECTION('center_axis',(-0.587785252292496,0.809016994374931,0.));
#121018=DIRECTION('ref_axis',(-0.809016994374931,-0.587785252292496,0.));
#121019=DIRECTION('center_axis',(0.587785252292471,-0.809016994374949,-8.27701011433315E-17));
#121020=DIRECTION('ref_axis',(0.809016994374949,0.587785252292471,6.81387014938251E-31));
#121021=DIRECTION('center_axis',(0.587785252292496,-0.809016994374931,6.42295984872268E-14));
#121022=DIRECTION('ref_axis',(0.809016994374931,0.587785252292496,4.46555866784231E-30));
#121023=DIRECTION('center_axis',(0.587785252292471,-0.809016994374949,-8.27701011433315E-17));
#121024=DIRECTION('ref_axis',(0.809016994374949,0.587785252292471,6.81387014938251E-31));
#121025=DIRECTION('center_axis',(-0.50901609747414,0.700659176689939,-0.499979330205134));
#121026=DIRECTION('ref_axis',(-0.293100449232374,0.405058175799812,0.866036951219467));
#121027=DIRECTION('center_axis',(0.293895658256105,-0.404512670528654,0.866022425483306));
#121028=DIRECTION('ref_axis',(4.45081872959523E-15,-0.906035197473508,-0.42320234042257));
#121029=DIRECTION('center_axis',(0.293895663527827,-0.404512677784641,0.866022420305062));
#121030=DIRECTION('ref_axis',(-0.809016994377093,-0.58778525228952,2.06309159991821E-12));
#121031=DIRECTION('center_axis',(-0.250002507183327,0.43301704446117,0.866022508719123));
#121032=DIRECTION('ref_axis',(0.866025403781571,0.500000000004967,-3.3219271679524E-12));
#121033=DIRECTION('center_axis',(-0.433035128829051,0.74997876016359,0.500012436348829));
#121034=DIRECTION('ref_axis',(0.249149002214356,-0.433518133177727,0.866017784402659));
#121035=DIRECTION('center_axis',(0.250002511507192,-0.433017051950268,-0.866022503726315));
#121036=DIRECTION('ref_axis',(-2.44740229890228E-15,0.894424794863789,-0.447218387740117));
#121037=DIRECTION('center_axis',(0.50000000000001,-0.866025403784433,0.));
#121038=DIRECTION('ref_axis',(0.866025403784433,0.50000000000001,0.));
#121039=DIRECTION('center_axis',(-0.499999999999998,0.86602540378444,7.0408453444955E-17));
#121040=DIRECTION('ref_axis',(-0.86602540378444,-0.499999999999998,-4.55018569865247E-33));
#121041=DIRECTION('center_axis',(-0.50000000000001,0.866025403784433,0.));
#121042=DIRECTION('ref_axis',(-0.866025403784433,-0.50000000000001,0.));
#121043=DIRECTION('center_axis',(-0.499999999999998,0.86602540378444,7.0408453444955E-17));
#121044=DIRECTION('ref_axis',(-0.86602540378444,-0.499999999999998,-4.55018569865247E-33));
#121045=DIRECTION('center_axis',(0.499999999999998,-0.86602540378444,0.));
#121046=DIRECTION('ref_axis',(0.86602540378444,0.499999999999998,0.));
#121047=DIRECTION('center_axis',(-0.264962106632886,0.458927830768629,-0.848045003637581));
#121048=DIRECTION('ref_axis',(4.53285787055483E-15,0.87947860205333,0.475938429348083));
#121049=DIRECTION('center_axis',(0.250002579266718,-0.43301716931321,0.866022425483292));
#121050=DIRECTION('ref_axis',(-2.13567853825987E-15,-0.89442473021642,-0.447218517033099));
#121051=DIRECTION('center_axis',(0.26496207377333,-0.458927817106627,0.848045021297503));
#121052=DIRECTION('ref_axis',(0.420286434054155,-0.736576463610279,-0.529919264233164));
#121053=DIRECTION('center_axis',(-0.264962078570523,0.45892778216319,-0.848045038708655));
#121054=DIRECTION('ref_axis',(-5.22840048568667E-15,0.879478631391258,0.475938375135017));
#121055=DIRECTION('center_axis',(0.25000257708735,-0.433017186566276,0.866022417485778));
#121056=DIRECTION('ref_axis',(0.429067561974281,-0.752263934574464,-0.499999999999992));
#121057=DIRECTION('center_axis',(0.43304850946242,-0.749993105181578,0.499979330205231));
#121058=DIRECTION('ref_axis',(0.250824363783207,-0.432512586701642,-0.866036951219406));
#121059=DIRECTION('center_axis',(-0.866146626230631,-0.499789977759954,
0.));
#121060=DIRECTION('ref_axis',(0.499789977759954,-0.866146626230631,0.));
#121061=DIRECTION('center_axis',(-0.499999999999998,0.86602540378444,7.0408453444955E-17));
#121062=DIRECTION('ref_axis',(-0.86602540378444,-0.499999999999998,-4.55018569865247E-33));
#121063=DIRECTION('center_axis',(0.500000000000051,-0.866025403784409,0.));
#121064=DIRECTION('ref_axis',(0.866025403784409,0.500000000000051,0.));
#121065=DIRECTION('center_axis',(-7.04084534449556E-17,-1.21951018649011E-16,
-1.));
#121066=DIRECTION('ref_axis',(0.,1.,-1.12832121675104E-16));
#121067=DIRECTION('center_axis',(-0.865904130412286,-0.500209992837952,
0.));
#121068=DIRECTION('ref_axis',(0.500209992837952,-0.865904130412285,0.));
#121069=DIRECTION('center_axis',(0.264962338412812,-0.458928232223238,-0.848044713969298));
#121070=DIRECTION('ref_axis',(2.57596116508717E-15,0.879478359737724,-0.475938877118735));
#121071=DIRECTION('center_axis',(0.264962078570518,-0.458927782163196,0.848045038708653));
#121072=DIRECTION('ref_axis',(3.68379810748961E-15,-0.879478631391255,-0.475938375135022));
#121073=DIRECTION('center_axis',(0.264962376556172,-0.458928247861003,-0.84804469358928));
#121074=DIRECTION('ref_axis',(-0.420092076158454,0.736687329159001,-0.529919264233201));
#121075=DIRECTION('center_axis',(0.264962371077221,-0.458928288799652,-0.848044673146739));
#121076=DIRECTION('ref_axis',(-5.61404975480703E-15,0.87947832558851,-0.475938940222411));
#121077=DIRECTION('center_axis',(-0.264962073789195,0.458927817280317,-0.848045021198552));
#121078=DIRECTION('ref_axis',(0.42775071226884,-0.732266960573829,-0.52991926423321));
#121079=DIRECTION('center_axis',(0.264962106632913,-0.458927830768691,0.848045003637539));
#121080=DIRECTION('ref_axis',(6.83278157480275E-15,-0.879478602053292,-0.475938429348154));
#121081=DIRECTION('center_axis',(-0.86615446498511,-0.499776392786171,0.));
#121082=DIRECTION('ref_axis',(0.499776392786171,-0.86615446498511,0.));
#121083=DIRECTION('center_axis',(0.50000000000001,-0.866025403784433,1.36592399683214E-14));
#121084=DIRECTION('ref_axis',(0.866025403784433,0.50000000000001,3.78074180857848E-32));
#121085=DIRECTION('center_axis',(-7.04084534449556E-17,-1.21951018649011E-16,
-1.));
#121086=DIRECTION('ref_axis',(0.,1.,-1.20114286872534E-16));
#121087=DIRECTION('center_axis',(-0.865896284857144,-0.500223573885314,
1.9979245236123E-14));
#121088=DIRECTION('ref_axis',(0.500223573885314,-0.865896284857144,3.61209325582807E-28));
#121089=DIRECTION('center_axis',(0.499999999999998,-0.86602540378444,-7.0408453444955E-17));
#121090=DIRECTION('ref_axis',(0.86602540378444,0.499999999999998,-9.66189415760573E-31));
#121091=DIRECTION('center_axis',(0.432983094185433,-0.750008802378803,-0.50001243634926));
#121092=DIRECTION('ref_axis',(-0.250863215179511,0.432528431861373,-0.866017784402457));
#121093=DIRECTION('center_axis',(-0.264962371077247,0.458928288799648,0.848044673146733));
#121094=DIRECTION('ref_axis',(5.87156122999725E-15,-0.87947832558851,0.47593894022241));
#121095=DIRECTION('center_axis',(-0.250002513557899,0.433017035276017,0.866022511471556));
#121096=DIRECTION('ref_axis',(-0.436883602758814,0.747751775417836,-0.499999999999954));
#121097=DIRECTION('center_axis',(0.250002511507137,-0.433017051950172,-0.866022503726379));
#121098=DIRECTION('ref_axis',(-1.53955398992304E-15,0.894424794863842,-0.447218387740011));
#121099=DIRECTION('center_axis',(-0.264962376528112,0.458928247652971,0.848044693710625));
#121100=DIRECTION('ref_axis',(-0.427943903631055,0.732154074454021,-0.529919264233139));
#121101=DIRECTION('center_axis',(-0.264962338412751,0.458928232223239,0.848044713969316));
#121102=DIRECTION('ref_axis',(-5.96114674208875E-16,-0.879478359737728,
0.475938877118728));
#121103=DIRECTION('center_axis',(0.50000000000001,-0.866025403784433,7.46354751724617E-14));
#121104=DIRECTION('ref_axis',(0.866025403784433,0.50000000000001,5.01950811882019E-30));
#121105=DIRECTION('center_axis',(-0.499999999999998,0.86602540378444,0.));
#121106=DIRECTION('ref_axis',(-0.86602540378444,-0.499999999999998,0.));
#121107=DIRECTION('center_axis',(0.499999999999998,-0.86602540378444,-7.0408453444955E-17));
#121108=DIRECTION('ref_axis',(0.86602540378444,0.499999999999998,-4.74656639208921E-31));
#121109=DIRECTION('center_axis',(0.50000000000001,-0.866025403784433,4.73169952358149E-14));
#121110=DIRECTION('ref_axis',(0.866025403784433,0.50000000000001,9.25800991341574E-31));
#121111=DIRECTION('center_axis',(0.499999999999998,-0.86602540378444,-7.0408453444955E-17));
#121112=DIRECTION('ref_axis',(0.86602540378444,0.499999999999998,-4.74656639208921E-31));
#121113=DIRECTION('center_axis',(-0.43298882701923,0.750027562856223,-0.499979330205226));
#121114=DIRECTION('ref_axis',(-0.249154705657362,0.433476564270054,0.866036951219417));
#121115=DIRECTION('center_axis',(0.250002579266723,-0.433017169313219,0.866022425483285));
#121116=DIRECTION('ref_axis',(-4.93751510904469E-15,-0.894424730216415,
-0.447218517033108));
#121117=DIRECTION('center_axis',(0.250002583755585,-0.43301717708815,0.866022420299926));
#121118=DIRECTION('ref_axis',(-0.866025403781823,-0.500000000004529,-3.00721826427187E-12));
#121119=DIRECTION('center_axis',(-0.203370361061121,0.456777309665475,0.866022508724017));
#121120=DIRECTION('ref_axis',(0.91354545764447,0.406736643071602,2.62257407997201E-12));
#121121=DIRECTION('center_axis',(-0.352268789802114,0.791134794600335,0.500012436349378));
#121122=DIRECTION('ref_axis',(0.202469153705661,-0.457186437787129,0.866017784402393));
#121123=DIRECTION('center_axis',(0.203370364581923,-0.45677731757327,-0.866022503726308));
#121124=DIRECTION('ref_axis',(3.44850229257831E-15,0.8845070363821,-0.466526850878441));
#121125=DIRECTION('center_axis',(0.406736643075797,-0.913545457642603,0.));
#121126=DIRECTION('ref_axis',(0.913545457642603,0.406736643075797,0.));
#121127=DIRECTION('center_axis',(-0.406736643075798,0.913545457642602,5.72753959967194E-17));
#121128=DIRECTION('ref_axis',(-0.913545457642602,-0.406736643075798,-5.41935833849719E-34));
#121129=DIRECTION('center_axis',(-0.406736643075807,0.913545457642598,0.));
#121130=DIRECTION('ref_axis',(-0.913545457642598,-0.406736643075807,0.));
#121131=DIRECTION('center_axis',(-0.406736643075798,0.913545457642602,5.72753959967194E-17));
#121132=DIRECTION('ref_axis',(-0.913545457642602,-0.406736643075798,-5.41935833849719E-34));
#121133=DIRECTION('center_axis',(0.406736643075817,-0.913545457642594,0.));
#121134=DIRECTION('ref_axis',(0.913545457642593,0.406736643075817,0.));
#121135=DIRECTION('center_axis',(-0.215539595588311,0.484109857923781,-0.848045003637569));
#121136=DIRECTION('ref_axis',(2.23395688692736E-15,0.868458021515989,0.495762710240024));
#121137=DIRECTION('center_axis',(0.203370419702463,-0.456777441376072,0.866022425483297));
#121138=DIRECTION('ref_axis',(-6.45206232673447E-15,-0.88450696681206,-0.466526982779055));
#121139=DIRECTION('center_axis',(0.215539564334499,-0.484109840902877,0.848045021297505));
#121140=DIRECTION('ref_axis',(0.340990855180419,-0.776473315753921,-0.529919264233183));
#121141=DIRECTION('center_axis',(-0.215539572760312,0.484109806651254,-0.848045038708669));
#121142=DIRECTION('ref_axis',(2.33490112882762E-15,0.868458052949978,0.495762655175168));
#121143=DIRECTION('center_axis',(0.203370415729658,-0.456777458307689,0.866022417485779));
#121144=DIRECTION('ref_axis',(0.348084091917939,-0.792992726923577,-0.499999999999973));
#121145=DIRECTION('center_axis',(0.352280597670804,-0.791150459692759,0.499979330205397));
#121146=DIRECTION('ref_axis',(0.204240445633901,-0.456361522797458,-0.866036951219318));
#121147=DIRECTION('center_axis',(-0.913644062717548,-0.406515100163541,
0.));
#121148=DIRECTION('ref_axis',(0.406515100163541,-0.913644062717548,0.));
#121149=DIRECTION('center_axis',(-0.406736643075798,0.913545457642602,5.72753959967194E-17));
#121150=DIRECTION('ref_axis',(-0.913545457642602,-0.406736643075798,-5.41935833849719E-34));
#121151=DIRECTION('center_axis',(0.406736643075807,-0.913545457642598,0.));
#121152=DIRECTION('ref_axis',(0.913545457642598,0.406736643075807,0.));
#121153=DIRECTION('center_axis',(-8.35415108931911E-17,-1.28642645648559E-16,
-1.));
#121154=DIRECTION('ref_axis',(0.,1.,-1.12832121675104E-16));
#121155=DIRECTION('center_axis',(-0.913446798847332,-0.406958162070208,
0.));
#121156=DIRECTION('ref_axis',(0.406958162070208,-0.913446798847332,0.));
#121157=DIRECTION('center_axis',(0.215539784135028,-0.484110281406739,-0.848044713969325));
#121158=DIRECTION('ref_axis',(2.06854852506343E-15,0.868457761888277,-0.495763165045573));
#121159=DIRECTION('center_axis',(0.215539572760318,-0.484109806651269,0.848045038708658));
#121160=DIRECTION('ref_axis',(3.65071283929963E-15,-0.868458052949968,-0.495762655175186));
#121161=DIRECTION('center_axis',(0.215539820427322,-0.484110300949258,-0.848044693589304));
#121162=DIRECTION('ref_axis',(-0.340785973393802,0.776563258036676,-0.529919264233243));
#121163=DIRECTION('center_axis',(0.215539810706706,-0.484110341087606,-0.848044673146739));
#121164=DIRECTION('ref_axis',(-5.01178427115621E-15,0.868457725299272,-0.495763229140701));
#121165=DIRECTION('center_axis',(-0.215539564340934,0.484109841073328,-0.848045021198567));
#121166=DIRECTION('ref_axis',(0.348864709025402,-0.772967650158224,-0.529919264233237));
#121167=DIRECTION('center_axis',(0.215539595588311,-0.484109857923781,0.848045003637569));
#121168=DIRECTION('ref_axis',(-2.23395688692736E-15,-0.868458021515989,
-0.495762710240024));
#121169=DIRECTION('center_axis',(-0.913650438514067,-0.406500770236727,
-2.49595411736522E-14));
#121170=DIRECTION('ref_axis',(0.406500770236727,-0.913650438514067,-1.62456620638984E-28));
#121171=DIRECTION('center_axis',(0.406736643075807,-0.913545457642598,0.));
#121172=DIRECTION('ref_axis',(0.913545457642598,0.406736643075807,0.));
#121173=DIRECTION('center_axis',(-8.35415108931911E-17,-1.28642645648559E-16,
-1.));
#121174=DIRECTION('ref_axis',(0.,1.,-1.20114286872534E-16));
#121175=DIRECTION('center_axis',(-0.913440415876952,-0.406972488803039,
2.71806413419028E-15));
#121176=DIRECTION('ref_axis',(0.406972488803039,-0.913440415876953,-4.76606432941746E-29));
#121177=DIRECTION('center_axis',(0.406736643075798,-0.913545457642602,-5.72753959967194E-17));
#121178=DIRECTION('ref_axis',(0.913545457642602,0.406736643075798,-5.47412728233073E-31));
#121179=DIRECTION('center_axis',(0.352213899941388,-0.79115923314136,-0.500012436348591));
#121180=DIRECTION('ref_axis',(-0.2042774279645,0.456381342215308,-0.866017784402816));
#121181=DIRECTION('center_axis',(-0.215539810706709,0.484110341087599,0.848044673146742));
#121182=DIRECTION('ref_axis',(-3.47902836708183E-15,-0.868457725299276,
0.495763229140693));
#121183=DIRECTION('center_axis',(-0.203370368361164,0.456777301206146,0.86602251147154));
#121184=DIRECTION('ref_axis',(-0.356328964666388,0.789322284583287,-0.5));
#121185=DIRECTION('center_axis',(0.203370364581877,-0.456777317573194,-0.86602250372636));
#121186=DIRECTION('ref_axis',(-5.71178009095155E-16,0.884507036382143,-0.466526850878359));
#121187=DIRECTION('center_axis',(-0.215539820426654,0.484110300737056,0.84804469371061));
#121188=DIRECTION('ref_axis',(-0.349068641861699,0.772875576443818,-0.529919264233209));
#121189=DIRECTION('center_axis',(-0.21553978413504,0.484110281406731,0.848044713969326));
#121190=DIRECTION('ref_axis',(-4.09518441222106E-16,-0.868457761888281,
0.495763165045567));
#121191=DIRECTION('center_axis',(0.406736643075807,-0.913545457642598,0.));
#121192=DIRECTION('ref_axis',(0.913545457642598,0.406736643075807,0.));
#121193=DIRECTION('center_axis',(-0.406736643075797,0.913545457642603,0.));
#121194=DIRECTION('ref_axis',(-0.913545457642603,-0.406736643075797,0.));
#121195=DIRECTION('center_axis',(0.406736643075798,-0.913545457642602,-5.72753959967194E-17));
#121196=DIRECTION('ref_axis',(0.913545457642602,0.406736643075798,-5.47412728233073E-31));
#121197=DIRECTION('center_axis',(0.406736643075807,-0.913545457642598,4.99133465116398E-14));
#121198=DIRECTION('ref_axis',(0.913545457642598,0.406736643075807,-2.16629559445036E-31));
#121199=DIRECTION('center_axis',(0.406736643075798,-0.913545457642602,-5.72753959967194E-17));
#121200=DIRECTION('ref_axis',(0.913545457642602,0.406736643075798,-5.47412728233073E-31));
#121201=DIRECTION('center_axis',(-0.352217640366552,0.79117849009073,-0.49997933020513));
#121202=DIRECTION('ref_axis',(-0.202479170978456,0.457145692796473,0.866036951219467));
#121203=DIRECTION('center_axis',(0.20337041970247,-0.456777441376074,0.866022425483294));
#121204=DIRECTION('ref_axis',(2.38658905335212E-15,-0.884506966812058,-0.46652698277906));
#121205=DIRECTION('center_axis',(0.203370423351772,-0.456777449572533,0.866022420303154));
#121206=DIRECTION('ref_axis',(-0.913545457644961,-0.4067366430705,3.35689480664158E-12));
#121207=DIRECTION('center_axis',(-0.154510046710301,0.475533027088488,0.866022508722285));
#121208=DIRECTION('ref_axis',(0.951056516295949,0.309016994372499,1.50360913918416E-12));
#121209=DIRECTION('center_axis',(-0.267642920195437,0.823622990673084,0.500012436349322));
#121210=DIRECTION('ref_axis',(0.153571010753323,-0.475845712132491,0.866017784402448));
#121211=DIRECTION('center_axis',(0.154510049384272,-0.475533035318153,-0.866022503726303));
#121212=DIRECTION('ref_axis',(-5.19003034006092E-15,0.876548788012428,-0.481313018974081));
#121213=DIRECTION('center_axis',(0.309016994374956,-0.951056516295151,-5.19628367180438E-14));
#121214=DIRECTION('ref_axis',(0.951056516295151,0.309016994374956,-4.37244376738262E-28));
#121215=DIRECTION('center_axis',(-0.309016994374945,0.951056516295154,4.35148173242966E-17));
#121216=DIRECTION('ref_axis',(-0.951056516295154,-0.309016994374945,1.82501959765721E-33));
#121217=DIRECTION('center_axis',(-0.309016994374964,0.951056516295148,4.35209621571297E-14));
#121218=DIRECTION('ref_axis',(-0.951056516295148,-0.309016994374964,3.68292735906465E-28));
#121219=DIRECTION('center_axis',(-0.309016994374945,0.951056516295154,4.35148173242966E-17));
#121220=DIRECTION('ref_axis',(-0.951056516295154,-0.309016994374945,1.82501959765721E-33));
#121221=DIRECTION('center_axis',(0.309016994374972,-0.951056516295146,0.));
#121222=DIRECTION('ref_axis',(0.951056516295146,0.309016994374972,0.));
#121223=DIRECTION('center_axis',(-0.163755587629913,0.503987876169014,-0.84804500363756));
#121224=DIRECTION('ref_axis',(1.56016625491565E-15,0.85964946204147,0.510884333691895));
#121225=DIRECTION('center_axis',(0.154510091261934,-0.475533164204412,0.866022425483295));
#121226=DIRECTION('ref_axis',(-2.58053144970935E-15,-0.876548714628837,
-0.481313152617434));
#121227=DIRECTION('center_axis',(0.163755558325956,-0.503987855974596,0.848045021297504));
#121228=DIRECTION('ref_axis',(0.257959309140313,-0.807862963764521,-0.5299192642332));
#121229=DIRECTION('center_axis',(-0.16375557028641,0.5039878227912,-0.848045038708652));
#121230=DIRECTION('ref_axis',(-1.11721014982679E-15,0.859649495083705,0.51088427809273));
#121231=DIRECTION('center_axis',(0.154510085544824,-0.475533180626773,0.866022417485781));
#121232=DIRECTION('ref_axis',(0.263286939714861,-0.825033325009131,-0.499999999999961));
#121233=DIRECTION('center_axis',(0.267653025932118,-0.823639804208658,0.499979330205263));
#121234=DIRECTION('ref_axis',(0.15541882643006,-0.475210466544791,-0.866036951219395));
#121235=DIRECTION('center_axis',(-0.951131423661017,-0.308786358060986,
0.));
#121236=DIRECTION('ref_axis',(0.308786358060986,-0.951131423661017,0.));
#121237=DIRECTION('center_axis',(-0.309016994374945,0.951056516295154,4.35148173242966E-17));
#121238=DIRECTION('ref_axis',(-0.951056516295154,-0.309016994374945,1.82501959765721E-33));
#121239=DIRECTION('center_axis',(0.309016994374922,-0.951056516295162,0.));
#121240=DIRECTION('ref_axis',(0.951056516295162,0.309016994374922,0.));
#121241=DIRECTION('center_axis',(-9.73020895656139E-17,-1.33924836902177E-16,
-1.));
#121242=DIRECTION('ref_axis',(0.,1.,-1.12832121675104E-16));
#121243=DIRECTION('center_axis',(-0.95098155300316,-0.309247612517378,0.));
#121244=DIRECTION('ref_axis',(0.309247612517378,-0.95098155300316,0.));
#121245=DIRECTION('center_axis',(0.163755730877736,-0.50398831704057,-0.848044713969324));
#121246=DIRECTION('ref_axis',(-1.7259771747372E-15,0.859649189130473,-0.510884792910613));
#121247=DIRECTION('center_axis',(0.163755570286409,-0.503987822791198,0.848045038708653));
#121248=DIRECTION('ref_axis',(1.48111944464757E-15,-0.859649495083707,-0.510884278092728));
#121249=DIRECTION('center_axis',(0.163755764936523,-0.503988340267036,-0.848044693589278));
#121250=DIRECTION('ref_axis',(-0.257746148173802,0.8079309973606,-0.529919264233218));
#121251=DIRECTION('center_axis',(0.163755751065515,-0.503988379172001,-0.848044673146732));
#121252=DIRECTION('ref_axis',(1.54456827304165E-15,0.859649150669465,-0.510884857627692));
#121253=DIRECTION('center_axis',(-0.163755558314028,0.503987856144943,-0.848045021198572));
#121254=DIRECTION('ref_axis',(0.266156471017446,-0.805199544417445,-0.529919264233221));
#121255=DIRECTION('center_axis',(0.1637555876299,-0.503987876168974,0.848045003637586));
#121256=DIRECTION('ref_axis',(-1.26854127671567E-15,-0.859649462041495,
-0.510884333691853));
#121257=DIRECTION('center_axis',(-0.951136266645027,-0.308771440182801,
9.11326423007149E-15));
#121258=DIRECTION('ref_axis',(0.308771440182801,-0.951136266645027,3.37083122818363E-29));
#121259=DIRECTION('center_axis',(0.309016994374964,-0.951056516295148,5.19628367180436E-14));
#121260=DIRECTION('ref_axis',(0.951056516295148,0.309016994374964,4.44026606255851E-28));
#121261=DIRECTION('center_axis',(-9.73020895656139E-17,-1.33924836902177E-16,
-1.));
#121262=DIRECTION('ref_axis',(0.,1.,-1.20114286872534E-16));
#121263=DIRECTION('center_axis',(-0.950976702550722,-0.309262527968967,
9.08207363789511E-15));
#121264=DIRECTION('ref_axis',(0.309262527968967,-0.950976702550722,-3.06533934379229E-29));
#121265=DIRECTION('center_axis',(0.309016994374945,-0.951056516295154,-4.35148173242966E-17));
#121266=DIRECTION('ref_axis',(0.951056516295154,0.309016994374945,1.86718128389415E-31));
#121267=DIRECTION('center_axis',(0.267585776504499,-0.823641557783651,-0.500012436349542));
#121268=DIRECTION('ref_axis',(-0.155453534481129,0.475234043094898,-0.866017784402261));
#121269=DIRECTION('center_axis',(-0.163755751065466,0.503988379172,0.848044673146743));
#121270=DIRECTION('ref_axis',(-4.67841503723397E-16,-0.859649150669469,
0.510884857627686));
#121271=DIRECTION('center_axis',(-0.154510054857217,0.475533019434505,0.866022511471568));
#121272=DIRECTION('ref_axis',(-0.271870311893668,0.822244813611426,-0.499999999999951));
#121273=DIRECTION('center_axis',(0.154510049384245,-0.475533035318,-0.866022503726391));
#121274=DIRECTION('ref_axis',(-2.49680260156733E-15,0.876548788012514,-0.481313018973924));
#121275=DIRECTION('center_axis',(-0.163755764952581,0.503988340057641,0.848044693710619));
#121276=DIRECTION('ref_axis',(-0.266368911015747,0.805129291877293,-0.529919264233198));
#121277=DIRECTION('center_axis',(-0.16375573087769,0.503988317040577,0.848044713969329));
#121278=DIRECTION('ref_axis',(1.0945036666319E-15,-0.859649189130472,0.510884792910616));
#121279=DIRECTION('center_axis',(0.309016994374964,-0.951056516295148,-8.44187456091391E-15));
#121280=DIRECTION('ref_axis',(0.951056516295148,0.309016994374964,-7.18667850250016E-29));
#121281=DIRECTION('center_axis',(-0.309016994374964,0.951056516295148,0.));
#121282=DIRECTION('ref_axis',(-0.951056516295148,-0.309016994374964,0.));
#121283=DIRECTION('center_axis',(0.309016994374945,-0.951056516295154,-4.35148173242966E-17));
#121284=DIRECTION('ref_axis',(0.951056516295154,0.309016994374945,1.86718128389415E-31));
#121285=DIRECTION('center_axis',(0.309016994374964,-0.951056516295148,6.88465858398714E-14));
#121286=DIRECTION('ref_axis',(0.951056516295148,0.309016994374964,5.83027010874528E-28));
#121287=DIRECTION('center_axis',(0.309016994374945,-0.951056516295154,-4.35148173242966E-17));
#121288=DIRECTION('ref_axis',(0.951056516295154,0.309016994374945,1.86718128389415E-31));
#121289=DIRECTION('center_axis',(-0.26758748354017,0.823661100222697,-0.499979330205336));
#121290=DIRECTION('ref_axis',(-0.153585232129532,0.475806237448003,0.866036951219342));
#121291=DIRECTION('center_axis',(0.154510091261981,-0.475533164204417,0.866022425483283));
#121292=DIRECTION('ref_axis',(-4.11550578150327E-15,-0.876548714628833,
-0.481313152617442));
#121293=DIRECTION('center_axis',(0.154510094034046,-0.475533172736068,0.866022420303978));
#121294=DIRECTION('ref_axis',(-0.951056516294272,-0.309016994377662,-1.67844740330627E-12));
#121295=DIRECTION('center_axis',(-0.103956887953752,0.489078705154832,0.866022508720786));
#121296=DIRECTION('ref_axis',(0.978147600734425,0.207911690814845,1.74838271998191E-12));
#121297=DIRECTION('center_axis',(-0.180084698747213,0.847087400905701,0.500012436349287));
#121298=DIRECTION('ref_axis',(0.102990311637667,-0.489291521291171,0.866017784402461));
#121299=DIRECTION('center_axis',(0.103956889752271,-0.489078713616369,-0.866022503726313));
#121300=DIRECTION('ref_axis',(-2.07612945625426E-15,0.870740345484704,-0.491743073916836));
#121301=DIRECTION('center_axis',(0.20791169081776,-0.978147600733806,5.34430112114423E-14));
#121302=DIRECTION('ref_axis',(0.978147600733806,0.20791169081776,-1.51620216886627E-28));
#121303=DIRECTION('center_axis',(-0.207911690817756,0.978147600733806,2.92774812072079E-17));
#121304=DIRECTION('ref_axis',(-0.978147600733806,-0.207911690817756,7.12388199405101E-34));
#121305=DIRECTION('center_axis',(-0.207911690817757,0.978147600733806,0.));
#121306=DIRECTION('ref_axis',(-0.978147600733806,-0.207911690817757,0.));
#121307=DIRECTION('center_axis',(-0.207911690817756,0.978147600733806,2.92774812072079E-17));
#121308=DIRECTION('ref_axis',(-0.978147600733806,-0.207911690817756,2.97300070454562E-33));
#121309=DIRECTION('center_axis',(0.207911690817754,-0.978147600733807,0.));
#121310=DIRECTION('ref_axis',(0.978147600733807,0.207911690817754,0.));
#121311=DIRECTION('center_axis',(-0.110177439185354,0.518344097776653,-0.848045003637581));
#121312=DIRECTION('ref_axis',(3.05434332738335E-15,0.853239582811869,0.521519140898039));
#121313=DIRECTION('center_axis',(0.103956917928293,-0.489078846174039,0.866022425483267));
#121314=DIRECTION('ref_axis',(-2.14699126507327E-16,-0.870740269393755,
-0.491743208652739));
#121315=DIRECTION('center_axis',(0.110177412155606,-0.518344074629213,0.848045021297501));
#121316=DIRECTION('ref_axis',(0.172101506940156,-0.830401496086937,-0.529919264233246));
#121317=DIRECTION('center_axis',(-0.110177427516371,0.518344042878406,-0.848045038708643));
#121318=DIRECTION('ref_axis',(-2.82117091702483E-16,0.853239616987298,0.521519084984786));
#121319=DIRECTION('center_axis',(0.103956910522966,-0.489078861909437,0.866022417485766));
#121320=DIRECTION('ref_axis',(0.175605160701873,-0.848034685337139,-0.500000000000009));
#121321=DIRECTION('center_axis',(0.180092991630808,-0.847105178671968,0.499979330205358));
#121322=DIRECTION('ref_axis',(0.104894406056248,-0.488852904973306,-0.866036951219327));
#121323=DIRECTION('center_axis',(-0.978197989689806,-0.20767448800183,0.));
#121324=DIRECTION('ref_axis',(0.20767448800183,-0.978197989689806,0.));
#121325=DIRECTION('center_axis',(-0.207911690817756,0.978147600733806,2.92774812072079E-17));
#121326=DIRECTION('ref_axis',(-0.978147600733806,-0.207911690817756,7.12388199405101E-34));
#121327=DIRECTION('center_axis',(0.207911690817757,-0.978147600733806,0.));
#121328=DIRECTION('ref_axis',(0.978147600733806,0.207911690817757,0.));
#121329=DIRECTION('center_axis',(-1.11539425682703E-16,-1.37739719617122E-16,
-1.));
#121330=DIRECTION('ref_axis',(0.,1.,-1.12832121675104E-16));
#121331=DIRECTION('center_axis',(-0.978097154258596,-0.208148881407602,
0.));
#121332=DIRECTION('ref_axis',(0.208148881407602,-0.978097154258596,0.));
#121333=DIRECTION('center_axis',(0.110177535564839,-0.518344551206567,-0.848044713969329));
#121334=DIRECTION('ref_axis',(2.56145575730607E-15,0.853239300541051,-0.521519602711363));
#121335=DIRECTION('center_axis',(0.110177427516339,-0.518344042878476,0.848045038708604));
#121336=DIRECTION('ref_axis',(-3.25887323275919E-16,-0.853239616987256,
-0.521519084984855));
#121337=DIRECTION('center_axis',(0.110177567011331,-0.518344577865485,-0.848044693589268));
#121338=DIRECTION('ref_axis',(-0.171882402211984,0.830446875606389,-0.529919264233171));
#121339=DIRECTION('center_axis',(0.110177549147492,-0.518344615107839,-0.848044673146738));
#121340=DIRECTION('ref_axis',(3.51301149947466E-15,0.853239260760973,-0.5215196677941));
#121341=DIRECTION('center_axis',(-0.110177412122692,0.518344074798062,-0.848045021198573));
#121342=DIRECTION('ref_axis',(0.180532167016074,-0.82860950396856,-0.529919264233202));
#121343=DIRECTION('center_axis',(0.110177439185352,-0.518344097776644,0.848045003637587));
#121344=DIRECTION('ref_axis',(-1.85242200733935E-15,-0.853239582811874,
-0.52151914089803));
#121345=DIRECTION('center_axis',(-0.978201246800567,-0.207659145615639,
2.01562116103772E-15));
#121346=DIRECTION('ref_axis',(0.207659145615639,-0.978201246800567,-8.39542909145296E-30));
#121347=DIRECTION('center_axis',(0.207911690817757,-0.978147600733806,0.));
#121348=DIRECTION('ref_axis',(0.978147600733806,0.207911690817757,0.));
#121349=DIRECTION('center_axis',(-1.11539425682703E-16,-1.37739719617122E-16,
-1.));
#121350=DIRECTION('ref_axis',(0.,1.,-1.20114286872534E-16));
#121351=DIRECTION('center_axis',(-0.978093889466682,-0.208164222161104,
0.));
#121352=DIRECTION('ref_axis',(0.208164222161104,-0.978093889466682,0.));
#121353=DIRECTION('center_axis',(0.207911690817756,-0.978147600733806,-2.92774812072079E-17));
#121354=DIRECTION('ref_axis',(0.978147600733806,0.207911690817756,2.34344808075099E-32));
#121355=DIRECTION('center_axis',(0.180025927305188,-0.847099893161506,-0.50001243634901));
#121356=DIRECTION('ref_axis',(-0.10492645948944,0.488879980360625,-0.86601778440261));
#121357=DIRECTION('center_axis',(-0.110177549147462,0.51834461510784,0.848044673146742));
#121358=DIRECTION('ref_axis',(-3.39955805632352E-15,-0.853239260760973,
0.521519667794099));
#121359=DIRECTION('center_axis',(-0.103956896856937,0.489078698391551,0.866022511471557));
#121360=DIRECTION('ref_axis',(-0.184432991092221,0.84615865639774,-0.499999999999948));
#121361=DIRECTION('center_axis',(0.103956889752284,-0.489078713616333,-0.866022503726332));
#121362=DIRECTION('ref_axis',(-1.29450859536298E-15,0.870740345484724,-0.491743073916801));
#121363=DIRECTION('center_axis',(-0.110177567041078,0.518344577660644,0.848044693710607));
#121364=DIRECTION('ref_axis',(-0.180750786618421,0.828561842309514,-0.529919264233229));
#121365=DIRECTION('center_axis',(-0.110177535564859,0.518344551206575,0.848044713969322));
#121366=DIRECTION('ref_axis',(-5.71220637831577E-16,-0.853239300541045,
0.521519602711372));
#121367=DIRECTION('center_axis',(0.207911690817757,-0.978147600733806,0.));
#121368=DIRECTION('ref_axis',(0.978147600733806,0.207911690817757,0.));
#121369=DIRECTION('center_axis',(-0.207911690817754,0.978147600733807,0.));
#121370=DIRECTION('ref_axis',(-0.978147600733807,-0.207911690817754,0.));
#121371=DIRECTION('center_axis',(0.207911690817756,-0.978147600733806,-2.92774812072079E-17));
#121372=DIRECTION('ref_axis',(0.978147600733806,0.207911690817756,2.34344808075099E-32));
#121373=DIRECTION('center_axis',(0.207911690817757,-0.978147600733806,8.51974703129737E-15));
#121374=DIRECTION('ref_axis',(0.978147600733806,0.207911690817757,3.738030205808E-32));
#121375=DIRECTION('center_axis',(0.207911690817756,-0.978147600733806,-2.92774812072079E-17));
#121376=DIRECTION('ref_axis',(0.978147600733806,0.207911690817756,2.34344808075099E-32));
#121377=DIRECTION('center_axis',(-0.180025582247462,0.847119506978757,-0.499979330205289));
#121378=DIRECTION('ref_axis',(-0.10300858135653,0.489253749387328,0.866036951219379));
#121379=DIRECTION('center_axis',(0.103956917928286,-0.489078846174001,0.866022425483289));
#121380=DIRECTION('ref_axis',(-6.13614011915674E-16,-0.870740269393776,
-0.491743208652701));
#121381=DIRECTION('center_axis',(0.103956919793741,-0.489078854950233,0.866022420303058));
#121382=DIRECTION('ref_axis',(-0.978147600733392,-0.207911690819706,-1.11896493554894E-12));
#121383=DIRECTION('center_axis',(-0.052264755777721,0.497265934580226,0.866022508719923));
#121384=DIRECTION('ref_axis',(0.994521895368293,0.104528463267463,1.04902963199238E-13));
#121385=DIRECTION('center_axis',(-0.0905534316534342,0.861270944310183,
0.50001243634817));
#121386=DIRECTION('ref_axis',(0.0512812291175601,-0.497376550148614,0.866017784403101));
#121387=DIRECTION('center_axis',(0.0522647566818157,-0.497265943181917,
-0.866022503726311));
#121388=DIRECTION('ref_axis',(1.36013666080525E-16,0.867207748104378,-0.497946504785137));
#121389=DIRECTION('center_axis',(0.104528463267629,-0.994521895368276,0.));
#121390=DIRECTION('ref_axis',(0.994521895368276,0.104528463267629,0.));
#121391=DIRECTION('center_axis',(-0.10452846326765,0.994521895368274,1.47193748793062E-17));
#121392=DIRECTION('ref_axis',(-0.994521895368274,-0.10452846326765,-3.45914136257457E-34));
#121393=DIRECTION('center_axis',(-0.104528463267629,0.994521895368276,-7.13889681646191E-16));
#121394=DIRECTION('ref_axis',(-0.994521895368276,-0.104528463267629,5.1828952049124E-31));
#121395=DIRECTION('center_axis',(-0.10452846326765,0.994521895368274,1.47193748793062E-17));
#121396=DIRECTION('ref_axis',(-0.994521895368274,-0.10452846326765,-3.45914136257457E-34));
#121397=DIRECTION('center_axis',(0.104528463267629,-0.994521895368276,0.));
#121398=DIRECTION('ref_axis',(0.994521895368276,0.104528463267629,0.));
#121399=DIRECTION('center_axis',(-0.0553921636609753,0.527021232978588,
-0.848045003637593));
#121400=DIRECTION('ref_axis',(5.60271951820181E-16,0.849349030019393,0.527831625809894));
#121401=DIRECTION('center_axis',(0.0522647708473854,-0.497266077958573,
0.866022425483295));
#121402=DIRECTION('ref_axis',(4.11267918639886E-16,-0.867207670398082,-0.497946640115918));
#121403=DIRECTION('center_axis',(0.0553921391946266,-0.527021207133024,
0.848045021297509));
#121404=DIRECTION('ref_axis',(0.0843581245662561,-0.843841975854613,-0.529919264233191));
#121405=DIRECTION('center_axis',(-0.0553921577943468,0.527021177161346,
-0.84804503870865));
#121406=DIRECTION('ref_axis',(-5.13852306535033E-16,0.84934906486752,0.527831569734768));
#121407=DIRECTION('center_axis',(0.0522647618447773,-0.49726609283302,0.866022417485766));
#121408=DIRECTION('ref_axis',(0.0859994148067042,-0.861744800189075,-0.499999999999996));
#121409=DIRECTION('center_axis',(0.0905598208269757,-0.861289491529615,
0.499979330205203));
#121410=DIRECTION('ref_axis',(0.0532207406005999,-0.497139368680954,-0.866036951219419));
#121411=DIRECTION('center_axis',(-0.994547213842469,-0.104287292793432,
6.79237952684971E-15));
#121412=DIRECTION('ref_axis',(0.104287292793432,-0.994547213842469,-7.19249397487602E-30));
#121413=DIRECTION('center_axis',(-0.10452846326765,0.994521895368274,1.47193748793062E-17));
#121414=DIRECTION('ref_axis',(-0.994521895368274,-0.10452846326765,-3.45914136257457E-34));
#121415=DIRECTION('center_axis',(0.104528463267628,-0.994521895368276,0.));
#121416=DIRECTION('ref_axis',(0.994521895368276,0.104528463267628,0.));
#121417=DIRECTION('center_axis',(-1.26097532010604E-16,-1.40045497140051E-16,
-1.));
#121418=DIRECTION('ref_axis',(0.,1.,-1.12832121675104E-16));
#121419=DIRECTION('center_axis',(-0.994496518411991,-0.10476962759516,0.));
#121420=DIRECTION('ref_axis',(0.10476962759516,-0.994496518411991,0.));
#121421=DIRECTION('center_axis',(0.0553922121161709,-0.527021693998982,
-0.848044713969329));
#121422=DIRECTION('ref_axis',(-1.55454699377472E-15,0.849348742192412,-0.527832088960275));
#121423=DIRECTION('center_axis',(0.0553921577943474,-0.527021177161352,
0.848045038708646));
#121424=DIRECTION('ref_axis',(1.53390223113159E-16,-0.849349064867516,-0.527831569734774));
#121425=DIRECTION('center_axis',(0.0553922405987001,-0.527021723799408,
-0.848044693589292));
#121426=DIRECTION('ref_axis',(-0.0841354767049436,0.843864204095777,-0.529919264233178));
#121427=DIRECTION('center_axis',(0.0553922189448978,-0.527021758969975,
-0.848044673146736));
#121428=DIRECTION('ref_axis',(-8.8709924467845E-16,0.849348701629309,-0.527832154231445));
#121429=DIRECTION('center_axis',(-0.0553921391437519,0.527021207297586,
-0.848045021198565));
#121430=DIRECTION('ref_axis',(0.092929914832894,-0.8429410443938,-0.529919264233186));
#121431=DIRECTION('center_axis',(0.0553921636609804,-0.527021232978636,
0.848045003637563));
#121432=DIRECTION('ref_axis',(4.3966219094204E-16,-0.849349030019363,-0.527831625809942));
#121433=DIRECTION('center_axis',(-0.994548849394383,-0.104271693993668,
0.));
#121434=DIRECTION('ref_axis',(0.104271693993668,-0.994548849394383,0.));
#121435=DIRECTION('center_axis',(0.104528463267629,-0.994521895368276,7.13889681646191E-16));
#121436=DIRECTION('ref_axis',(0.994521895368276,0.104528463267629,-5.1828952049124E-31));
#121437=DIRECTION('center_axis',(-1.26097532010604E-16,-1.40045497140051E-16,
-1.));
#121438=DIRECTION('ref_axis',(0.,1.,-1.20114286872534E-16));
#121439=DIRECTION('center_axis',(-0.994494875050338,-0.104785225574086,
-5.72514616500437E-15));
#121440=DIRECTION('ref_axis',(0.104785225574086,-0.994494875050338,8.5757403076988E-30));
#121441=DIRECTION('center_axis',(0.10452846326765,-0.994521895368274,-1.47193748793062E-17));
#121442=DIRECTION('ref_axis',(0.994521895368274,0.10452846326765,1.81599985181705E-32));
#121443=DIRECTION('center_axis',(0.0904936763735575,-0.861277224843726,
-0.500012436347226));
#121444=DIRECTION('ref_axis',(-0.0532497883641599,0.49716964623344,-0.866017784403581));
#121445=DIRECTION('center_axis',(-0.0553922189448982,0.527021758969983,
0.848044673146731));
#121446=DIRECTION('ref_axis',(3.87123138543772E-16,-0.849348701629304,0.527832154231452));
#121447=DIRECTION('center_axis',(-0.0522647653346091,0.4972659287836,0.866022511471556));
#121448=DIRECTION('ref_axis',(-0.0949749838151956,0.860801807879908,-0.499999999999986));
#121449=DIRECTION('center_axis',(0.0522647566817756,-0.497265943181796,
-0.866022503726383));
#121450=DIRECTION('ref_axis',(-8.82337668496122E-16,0.867207748104448,-0.497946504785014));
#121451=DIRECTION('center_axis',(-0.055392240655012,0.527021723598282,0.848044693710605));
#121452=DIRECTION('ref_axis',(-0.0931523188089191,0.842916495801946,-0.529919264233232));
#121453=DIRECTION('center_axis',(-0.0553922121161263,0.527021693999001,
0.84804471396932));
#121454=DIRECTION('ref_axis',(3.59452935077625E-16,-0.849348742192401,0.527832088960293));
#121455=DIRECTION('center_axis',(0.104528463267629,-0.994521895368276,7.13889681646191E-16));
#121456=DIRECTION('ref_axis',(0.994521895368276,0.104528463267629,-5.1828952049124E-31));
#121457=DIRECTION('center_axis',(-0.104528463267628,0.994521895368276,0.));
#121458=DIRECTION('ref_axis',(-0.994521895368276,-0.104528463267628,0.));
#121459=DIRECTION('center_axis',(0.10452846326765,-0.994521895368274,-1.47193748793062E-17));
#121460=DIRECTION('ref_axis',(0.994521895368274,0.10452846326765,1.81599985181705E-32));
#121461=DIRECTION('center_axis',(0.104528463267629,-0.994521895368276,7.13889681646191E-16));
#121462=DIRECTION('ref_axis',(0.994521895368276,0.104528463267629,-5.1828952049124E-31));
#121463=DIRECTION('center_axis',(0.10452846326765,-0.994521895368274,-1.47193748793062E-17));
#121464=DIRECTION('ref_axis',(0.994521895368274,0.10452846326765,1.81599985181705E-32));
#121465=DIRECTION('center_axis',(-0.0904912830026993,0.861296695145209,
-0.499979330205226));
#121466=DIRECTION('ref_axis',(-0.0513033469913138,0.497340894869987,0.86603695121941));
#121467=DIRECTION('center_axis',(0.0522647708473846,-0.497266077958562,
0.866022425483301));
#121468=DIRECTION('ref_axis',(1.07940002356267E-15,-0.867207670398088,-0.497946640115907));
#121469=DIRECTION('center_axis',(0.0522647717852579,-0.49726608688173,0.866022420303058));
#121470=DIRECTION('ref_axis',(-0.994521895368593,-0.104528463264607,1.74838271179562E-12));
#121471=DIRECTION('center_axis',(1.82820803129159E-15,0.500005014362592,
0.866022508721491));
#121472=DIRECTION('ref_axis',(1.,7.55301335024178E-12,-4.37095679990844E-12));
#121473=DIRECTION('center_axis',(-3.00422155937779E-5,0.866018223015147,
0.50001243634849));
#121474=DIRECTION('ref_axis',(-0.000989701348168873,-0.500012217439953,
0.866017784402851));
#121475=DIRECTION('center_axis',(-1.99980824065794E-14,-0.500005023014372,
-0.866022503726316));
#121476=DIRECTION('ref_axis',(2.4869776260939E-28,0.866022503726316,-0.500005023014372));
#121477=DIRECTION('center_axis',(0.,-1.,0.));
#121478=DIRECTION('ref_axis',(0.,0.,-1.));
#121479=DIRECTION('center_axis',(3.49148133884313E-15,1.,-4.91659602599733E-31));
#121480=DIRECTION('ref_axis',(-1.,3.49148133884313E-15,-3.11150763893057E-61));
#121481=DIRECTION('center_axis',(0.,1.,0.));
#121482=DIRECTION('ref_axis',(0.,0.,1.));
#121483=DIRECTION('center_axis',(3.49148133884313E-15,1.,-4.91659602599733E-31));
#121484=DIRECTION('ref_axis',(-1.,3.49148133884313E-15,-3.11150763893057E-61));
#121485=DIRECTION('center_axis',(0.,-1.,0.));
#121486=DIRECTION('ref_axis',(0.,0.,-1.));
#121487=DIRECTION('center_axis',(0.,0.52992421326579,-0.848045003637563));
#121488=DIRECTION('ref_axis',(0.,0.848045003637563,0.52992421326579));
#121489=DIRECTION('center_axis',(0.,-0.500005158533422,0.866022425483294));
#121490=DIRECTION('ref_axis',(0.,-0.866022425483294,-0.500005158533421));
#121491=DIRECTION('center_axis',(-2.16272591755565E-8,-0.529924185004355,
0.848045021297496));
#121492=DIRECTION('ref_axis',(-0.00430950303426538,-0.848037146343315,-0.529919264233227));
#121493=DIRECTION('center_axis',(0.,0.529924157141051,-0.848045038708645));
#121494=DIRECTION('ref_axis',(0.,0.848045038708645,0.529924157141051));
#121495=DIRECTION('center_axis',(-1.05145777036886E-8,-0.500005172385382,
0.866022417485751));
#121496=DIRECTION('ref_axis',(-0.00454855868556522,-0.866013458679398,-0.50000000000003));
#121497=DIRECTION('center_axis',(3.4457674556699E-5,-0.866037336481604,
0.499979330205277));
#121498=DIRECTION('ref_axis',(0.000963977567656715,-0.499979069431795,-0.866036951219384));
#121499=DIRECTION('center_axis',(-0.999999970597889,0.000242495818334613,
1.33391011393658E-16));
#121500=DIRECTION('ref_axis',(-0.000242495818334613,-0.999999970597889,
-6.94884378066767E-34));
#121501=DIRECTION('center_axis',(3.49148133884313E-15,1.,-4.91659602599733E-31));
#121502=DIRECTION('ref_axis',(-1.,3.49148133884313E-15,-3.11150763893057E-61));
#121503=DIRECTION('center_axis',(0.,-1.,0.));
#121504=DIRECTION('ref_axis',(0.,0.,-1.));
#121505=DIRECTION('center_axis',(-1.40816906889911E-16,-1.40816906889911E-16,
-1.));
#121506=DIRECTION('ref_axis',(-1.,4.30611566690962E-33,1.12832121675104E-16));
#121507=DIRECTION('center_axis',(-0.999999970597889,-0.000242495818327663,
1.46730112533024E-16));
#121508=DIRECTION('ref_axis',(0.000242495818327663,-0.999999970597889,8.25475152210998E-34));
#121509=DIRECTION('center_axis',(2.89534733035821E-14,-0.529924676825566,
-0.848044713969328));
#121510=DIRECTION('ref_axis',(-3.85833700151325E-28,0.848044713969328,-0.529924676825566));
#121511=DIRECTION('center_axis',(-4.63346027506605E-14,-0.52992415714112,
0.848045038708602));
#121512=DIRECTION('ref_axis',(-2.08103008143499E-28,-0.848045038708602,
-0.52992415714112));
#121513=DIRECTION('center_axis',(2.5213841626272E-8,-0.529924709439993,
-0.848044693589281));
#121514=DIRECTION('ref_axis',(0.00453325469213716,0.848035979777049,-0.529919264233219));
#121515=DIRECTION('center_axis',(4.63345827774717E-14,-0.529924742154432,
-0.848044673146739));
#121516=DIRECTION('ref_axis',(-1.03497526951197E-27,0.848044673146739,-0.529924742154432));
#121517=DIRECTION('center_axis',(2.1691013480987E-8,0.529924185162642,-0.848045021198586));
#121518=DIRECTION('ref_axis',(0.00430950302060195,-0.848037146343406,-0.529919264233192));
#121519=DIRECTION('center_axis',(0.,-0.52992421326579,0.848045003637563));
#121520=DIRECTION('ref_axis',(0.,-0.848045003637563,-0.52992421326579));
#121521=DIRECTION('center_axis',(-0.99999996667151,0.000258180127967688,
1.60069213043906E-16));
#121522=DIRECTION('ref_axis',(-0.000258180127967688,-0.99999996667151,1.64102447194681E-33));
#121523=DIRECTION('center_axis',(0.,-1.,0.));
#121524=DIRECTION('ref_axis',(0.,0.,-1.));
#121525=DIRECTION('center_axis',(-1.40816906889911E-16,-1.40816906889911E-16,
-1.));
#121526=DIRECTION('ref_axis',(-1.,3.33384117180795E-33,1.20114286872534E-16));
#121527=DIRECTION('center_axis',(-0.99999996667151,-0.000258180127960702,
1.45963035752429E-16));
#121528=DIRECTION('ref_axis',(0.000258180127960701,-0.99999996667151,-2.00104120761843E-33));
#121529=DIRECTION('center_axis',(-3.49148133884313E-15,-1.,4.91659602599733E-31));
#121530=DIRECTION('ref_axis',(1.,-3.49148133884313E-15,3.17373779170918E-59));
#121531=DIRECTION('center_axis',(-3.00422140677667E-5,-0.866018223016196,
-0.500012436346673));
#121532=DIRECTION('ref_axis',(-0.000989701277811038,0.500012217438168,-0.866017784403962));
#121533=DIRECTION('center_axis',(0.,0.529924742154432,0.848044673146739));
#121534=DIRECTION('ref_axis',(0.,-0.848044673146739,0.529924742154432));
#121535=DIRECTION('center_axis',(-1.01121416634232E-8,0.500005009599418,
0.866022511471547));
#121536=DIRECTION('ref_axis',(-0.0044764107678598,0.866013834616202,-0.49999999999998));
#121537=DIRECTION('center_axis',(0.,-0.500005023014331,-0.86602250372634));
#121538=DIRECTION('ref_axis',(0.,0.86602250372634,-0.500005023014331));
#121539=DIRECTION('center_axis',(-2.52896301115931E-8,0.529924709245837,
0.848044693710606));
#121540=DIRECTION('ref_axis',(-0.00453325469037203,0.848035979777047,-0.529919264233237));
#121541=DIRECTION('center_axis',(0.,0.529924676825566,0.848044713969328));
#121542=DIRECTION('ref_axis',(0.,-0.848044713969328,0.529924676825566));
#121543=DIRECTION('center_axis',(0.,-1.,0.));
#121544=DIRECTION('ref_axis',(0.,0.,-1.));
#121545=DIRECTION('center_axis',(0.,1.,0.));
#121546=DIRECTION('ref_axis',(0.,0.,1.));
#121547=DIRECTION('center_axis',(-3.49148133884313E-15,-1.,4.91659602599733E-31));
#121548=DIRECTION('ref_axis',(1.,-3.49148133884313E-15,3.17373779170918E-59));
#121549=DIRECTION('center_axis',(0.,-1.,0.));
#121550=DIRECTION('ref_axis',(0.,0.,-1.));
#121551=DIRECTION('center_axis',(-3.49148133884313E-15,-1.,4.91659602599733E-31));
#121552=DIRECTION('ref_axis',(1.,-3.49148133884313E-15,3.17373779170918E-59));
#121553=DIRECTION('center_axis',(3.4457674514454E-5,0.866037336481586,-0.499979330205309));
#121554=DIRECTION('ref_axis',(0.000963977569514902,0.499979069431826,0.866036951219364));
#121555=DIRECTION('center_axis',(0.,-0.500005158533422,0.866022425483294));
#121556=DIRECTION('ref_axis',(0.,-0.866022425483294,-0.500005158533421));
#121557=DIRECTION('center_axis',(-1.43938253461657E-15,-0.500005167509872,
0.866022420300667));
#121558=DIRECTION('ref_axis',(-1.,1.67844740333716E-12,9.79094318613344E-13));
#121559=DIRECTION('center_axis',(0.0522647557773262,0.497265934576325,0.866022508722187));
#121560=DIRECTION('ref_axis',(0.994521895368361,-0.104528463266816,-4.89547161592758E-13));
#121561=DIRECTION('center_axis',(0.090493676372036,0.861277224842593,0.500012436349452));
#121562=DIRECTION('ref_axis',(-0.0532497883447732,-0.497169646237728,0.866017784402312));
#121563=DIRECTION('center_axis',(-0.0522647566818161,-0.497265943181921,
-0.866022503726309));
#121564=DIRECTION('ref_axis',(1.04964660243371E-15,0.867207748104375,-0.497946504785141));
#121565=DIRECTION('center_axis',(-0.104528463267684,-0.99452189536827,0.));
#121566=DIRECTION('ref_axis',(0.99452189536827,-0.104528463267684,0.));
#121567=DIRECTION('center_axis',(0.104528463267657,0.994521895368273,-1.47193748793071E-17));
#121568=DIRECTION('ref_axis',(-0.994521895368273,0.104528463267657,6.90194618736947E-35));
#121569=DIRECTION('center_axis',(0.104528463267683,0.99452189536827,0.));
#121570=DIRECTION('ref_axis',(-0.99452189536827,0.104528463267683,0.));
#121571=DIRECTION('center_axis',(0.104528463267657,0.994521895368273,-1.47193748793071E-17));
#121572=DIRECTION('ref_axis',(-0.994521895368273,0.104528463267657,6.90194618736947E-35));
#121573=DIRECTION('center_axis',(-0.104528463267683,-0.99452189536827,0.));
#121574=DIRECTION('ref_axis',(0.99452189536827,-0.104528463267683,0.));
#121575=DIRECTION('center_axis',(0.0553921636610116,0.527021232978657,-0.848045003637547));
#121576=DIRECTION('ref_axis',(-1.00433790736153E-15,0.849349030019349,0.527831625809965));
#121577=DIRECTION('center_axis',(-0.0522647708473925,-0.49726607795856,
0.866022425483302));
#121578=DIRECTION('ref_axis',(-1.15905889347861E-15,-0.867207670398089,
-0.497946640115906));
#121579=DIRECTION('center_axis',(-0.055392182216939,-0.527021202611195,
0.84804502129751));
#121580=DIRECTION('ref_axis',(-0.0929299148227876,-0.842941044394903,-0.529919264233203));
#121581=DIRECTION('center_axis',(0.0553921577943745,0.527021177161334,-0.848045038708656));
#121582=DIRECTION('ref_axis',(1.26600207161536E-15,0.849349064867527,0.527831569734757));
#121583=DIRECTION('center_axis',(-0.0522647827511113,-0.497266090635737,
0.866022417485731));
#121584=DIRECTION('ref_axis',(-0.0950466972058103,-0.860793892491238,-0.500000000000051));
#121585=DIRECTION('center_axis',(-0.0904912830032905,-0.861296695145041,
0.499979330205408));
#121586=DIRECTION('ref_axis',(-0.0513033469918369,-0.497340894870115,-0.866036951219305));
#121587=DIRECTION('center_axis',(-0.994496518411991,0.10476962759516,0.));
#121588=DIRECTION('ref_axis',(-0.10476962759516,-0.994496518411991,0.));
#121589=DIRECTION('center_axis',(0.104528463267657,0.994521895368273,-1.47193748793071E-17));
#121590=DIRECTION('ref_axis',(-0.994521895368273,0.104528463267657,6.90194618736947E-35));
#121591=DIRECTION('center_axis',(-0.104528463267683,-0.99452189536827,0.));
#121592=DIRECTION('ref_axis',(0.99452189536827,-0.104528463267683,0.));
#121593=DIRECTION('center_axis',(-1.55536281769218E-16,-1.40045497140051E-16,
-1.));
#121594=DIRECTION('ref_axis',(-1.,6.26344097005036E-33,1.12832121675104E-16));
#121595=DIRECTION('center_axis',(-0.994547213842468,0.104287292793436,0.));
#121596=DIRECTION('ref_axis',(-0.104287292793436,-0.994547213842468,0.));
#121597=DIRECTION('center_axis',(-0.0553922121162014,-0.527021693998993,
-0.84804471396932));
#121598=DIRECTION('ref_axis',(7.7366740613734E-16,0.849348742192405,-0.527832088960287));
#121599=DIRECTION('center_axis',(-0.0553921577943754,-0.527021177161343,
0.84804503870865));
#121600=DIRECTION('ref_axis',(-6.73068733579088E-16,-0.849349064867521,
-0.527831569734766));
#121601=DIRECTION('center_axis',(-0.0553921904483075,-0.527021729070454,
-0.848044693589275));
#121602=DIRECTION('ref_axis',(0.0931523188238882,0.842916495800322,-0.529919264233183));
#121603=DIRECTION('center_axis',(-0.0553922189449272,-0.527021758969979,
-0.848044673146731));
#121604=DIRECTION('ref_axis',(5.44485983564514E-16,0.849348701629306,-0.52783215423145));
#121605=DIRECTION('center_axis',(0.055392182295534,0.52702120276216,-0.848045021198559));
#121606=DIRECTION('ref_axis',(-0.0843581245707786,-0.843841975854142,-0.529919264233221));
#121607=DIRECTION('center_axis',(-0.0553921636610064,-0.527021232978609,
0.848045003637578));
#121608=DIRECTION('ref_axis',(-5.90605431002811E-16,-0.84934903001938,-0.527831625809916));
#121609=DIRECTION('center_axis',(-0.994494875050338,0.10478522557409,0.));
#121610=DIRECTION('ref_axis',(-0.10478522557409,-0.994494875050338,0.));
#121611=DIRECTION('center_axis',(-0.104528463267683,-0.99452189536827,0.));
#121612=DIRECTION('ref_axis',(0.99452189536827,-0.104528463267683,0.));
#121613=DIRECTION('center_axis',(-1.55536281769218E-16,-1.40045497140051E-16,
-1.));
#121614=DIRECTION('ref_axis',(-1.,5.41749190418792E-33,1.20114286872534E-16));
#121615=DIRECTION('center_axis',(-0.994548849394382,0.104271693993676,0.));
#121616=DIRECTION('ref_axis',(-0.104271693993676,-0.994548849394382,0.));
#121617=DIRECTION('center_axis',(-0.104528463267657,-0.994521895368273,
1.47193748793071E-17));
#121618=DIRECTION('ref_axis',(0.994521895368273,-0.104528463267657,1.77461199646142E-32));
#121619=DIRECTION('center_axis',(-0.0905534316536479,-0.861270944310105,
-0.500012436348265));
#121620=DIRECTION('ref_axis',(0.0512812290951098,0.497376550151059,-0.866017784403026));
#121621=DIRECTION('center_axis',(0.0553922189449268,0.527021758969972,0.848044673146736));
#121622=DIRECTION('ref_axis',(-1.02650725247837E-15,-0.84934870162931,0.527832154231442));
#121623=DIRECTION('center_axis',(0.0522647452194355,0.497265930897802,0.86602251147155));
#121624=DIRECTION('ref_axis',(0.086071206774765,0.861737632556662,-0.499999999999975));
#121625=DIRECTION('center_axis',(-0.0522647566818046,-0.497265943181812,
-0.866022503726373));
#121626=DIRECTION('ref_axis',(-1.28065569756335E-16,0.867207748104438,-0.497946504785031));
#121627=DIRECTION('center_axis',(0.0553921903445286,0.527021728886068,0.848044693710641));
#121628=DIRECTION('ref_axis',(0.084135476695041,0.843864204096788,-0.52991926423314));
#121629=DIRECTION('center_axis',(0.0553922121161999,0.527021693998978,0.848044713969329));
#121630=DIRECTION('ref_axis',(-1.1898461170849E-16,-0.849348742192414,0.527832088960272));
#121631=DIRECTION('center_axis',(-0.104528463267683,-0.99452189536827,0.));
#121632=DIRECTION('ref_axis',(0.99452189536827,-0.104528463267683,0.));
#121633=DIRECTION('center_axis',(0.104528463267682,0.99452189536827,0.));
#121634=DIRECTION('ref_axis',(-0.99452189536827,0.104528463267682,0.));
#121635=DIRECTION('center_axis',(-0.104528463267657,-0.994521895368273,
1.47193748793071E-17));
#121636=DIRECTION('ref_axis',(0.994521895368273,-0.104528463267657,1.77461199646142E-32));
#121637=DIRECTION('center_axis',(-0.104528463267683,-0.99452189536827,-5.50515425719855E-14));
#121638=DIRECTION('ref_axis',(0.99452189536827,-0.104528463267683,-6.20682976726545E-31));
#121639=DIRECTION('center_axis',(-0.104528463267657,-0.994521895368273,
1.47193748793071E-17));
#121640=DIRECTION('ref_axis',(0.994521895368273,-0.104528463267657,1.77461199646142E-32));
#121641=DIRECTION('center_axis',(0.0905598208272809,0.861289491529787,-0.499979330204851));
#121642=DIRECTION('ref_axis',(0.0532207405929829,0.497139368681404,0.866036951219629));
#121643=DIRECTION('center_axis',(-0.0522647708474152,-0.497266077958594,
0.866022425483281));
#121644=DIRECTION('ref_axis',(8.80735367310087E-16,-0.867207670398069,-0.49794664011594));
#121645=DIRECTION('center_axis',(-0.0522647717855183,-0.497266086884147,
0.866022420301654));
#121646=DIRECTION('ref_axis',(-0.994521895368054,0.104528463269739,1.1889002440261E-12));
#121647=DIRECTION('center_axis',(0.103956887953211,0.489078705152364,0.866022508722245));
#121648=DIRECTION('ref_axis',(0.978147600733814,-0.20791169081772,0.));
#121649=DIRECTION('center_axis',(0.180025927304861,0.847099893161487,0.500012436349159));
#121650=DIRECTION('ref_axis',(-0.104926459551779,-0.488879980347496,0.866017784402469));
#121651=DIRECTION('center_axis',(-0.103956889752312,-0.489078713616371,
-0.866022503726307));
#121652=DIRECTION('ref_axis',(1.59798216899832E-15,0.870740345484702,-0.49174307391684));
#121653=DIRECTION('center_axis',(-0.207911690817751,-0.978147600733807,
0.));
#121654=DIRECTION('ref_axis',(0.978147600733807,-0.207911690817751,0.));
#121655=DIRECTION('center_axis',(0.207911690817763,0.978147600733805,-2.92774812072088E-17));
#121656=DIRECTION('ref_axis',(-0.978147600733805,0.207911690817763,1.17770789928191E-33));
#121657=DIRECTION('center_axis',(0.207911690817757,0.978147600733806,-2.83991567709928E-15));
#121658=DIRECTION('ref_axis',(-0.978147600733806,0.207911690817757,9.97553654791534E-32));
#121659=DIRECTION('center_axis',(0.207911690817763,0.978147600733805,-2.92774812072088E-17));
#121660=DIRECTION('ref_axis',(-0.978147600733805,0.207911690817763,1.17770789928191E-33));
#121661=DIRECTION('center_axis',(-0.207911690817757,-0.978147600733806,
0.));
#121662=DIRECTION('ref_axis',(0.978147600733806,-0.207911690817757,0.));
#121663=DIRECTION('center_axis',(0.110177439185365,0.518344097776706,-0.848045003637548));
#121664=DIRECTION('ref_axis',(-1.70903056951593E-15,0.853239582811836,0.521519140898093));
#121665=DIRECTION('center_axis',(-0.103956917928266,-0.489078846174005,
0.86602242548329));
#121666=DIRECTION('ref_axis',(8.66848073542193E-16,-0.870740269393775,-0.491743208652703));
#121667=DIRECTION('center_axis',(-0.110177454465019,-0.518344065636052,
0.848045021297512));
#121668=DIRECTION('ref_axis',(-0.180532167030478,-0.828609503965439,-0.529919264233174));
#121669=DIRECTION('center_axis',(0.110177427516371,0.518344042878403,-0.848045038708645));
#121670=DIRECTION('ref_axis',(6.45685183168496E-16,0.8532396169873,0.521519084984783));
#121671=DIRECTION('center_axis',(-0.103956931089751,-0.489078857537854,
0.866022417485753));
#121672=DIRECTION('ref_axis',(-0.184503484221683,-0.846143288285166,-0.500000000000025));
#121673=DIRECTION('center_axis',(-0.180025582247593,-0.847119506978661,
0.499979330205405));
#121674=DIRECTION('ref_axis',(-0.103008581348147,-0.489253749389224,-0.866036951219305));
#121675=DIRECTION('center_axis',(-0.978097154258593,0.208148881407615,0.));
#121676=DIRECTION('ref_axis',(-0.208148881407615,-0.978097154258593,0.));
#121677=DIRECTION('center_axis',(0.207911690817763,0.978147600733805,-2.92774812072088E-17));
#121678=DIRECTION('ref_axis',(-0.978147600733805,0.207911690817763,1.17770789928191E-33));
#121679=DIRECTION('center_axis',(-0.207911690817757,-0.978147600733806,
0.));
#121680=DIRECTION('ref_axis',(0.978147600733806,-0.207911690817757,0.));
#121681=DIRECTION('center_axis',(-1.70094388097119E-16,-1.37739719617122E-16,
-1.));
#121682=DIRECTION('ref_axis',(-1.,-7.04637109130665E-33,2.25664243350207E-16));
#121683=DIRECTION('center_axis',(-0.978197989689808,0.20767448800182,0.));
#121684=DIRECTION('ref_axis',(-0.20767448800182,-0.978197989689808,0.));
#121685=DIRECTION('center_axis',(-0.110177535564866,-0.518344551206614,
-0.848044713969297));
#121686=DIRECTION('ref_axis',(-5.11710185561069E-16,0.853239300541021,-0.521519602711412));
#121687=DIRECTION('center_axis',(-0.110177427516374,-0.518344042878421,
0.848045038708634));
#121688=DIRECTION('ref_axis',(1.65648280181603E-15,-0.853239616987289,-0.521519084984801));
#121689=DIRECTION('center_axis',(-0.110177517687313,-0.518344588349581,
-0.848044693589297));
#121690=DIRECTION('ref_axis',(0.180750786622895,0.828561842308536,-0.529919264233231));
#121691=DIRECTION('center_axis',(-0.110177549147463,-0.51834461510784,-0.848044673146742));
#121692=DIRECTION('ref_axis',(-3.37087989426115E-15,0.853239260760974,-0.521519667794099));
#121693=DIRECTION('center_axis',(0.110177454561672,0.518344065777387,-0.848045021198568));
#121694=DIRECTION('ref_axis',(-0.172101506910798,-0.830401496093066,-0.529919264233176));
#121695=DIRECTION('center_axis',(-0.110177439185362,-0.51834409777669,0.848045003637558));
#121696=DIRECTION('ref_axis',(-3.31296850970174E-16,-0.853239582811845,
-0.521519140898077));
#121697=DIRECTION('center_axis',(-0.978093889466682,0.208164222161104,0.));
#121698=DIRECTION('ref_axis',(-0.208164222161104,-0.978093889466682,0.));
#121699=DIRECTION('center_axis',(-0.207911690817757,-0.978147600733806,
0.));
#121700=DIRECTION('ref_axis',(0.978147600733806,-0.207911690817757,0.));
#121701=DIRECTION('center_axis',(-1.70094388097119E-16,-1.37739719617122E-16,
-1.));
#121702=DIRECTION('ref_axis',(-1.,7.29277756332989E-33,1.20114286872534E-16));
#121703=DIRECTION('center_axis',(-0.978201246800563,0.207659145615656,0.));
#121704=DIRECTION('ref_axis',(-0.207659145615656,-0.978201246800563,0.));
#121705=DIRECTION('center_axis',(-0.207911690817763,-0.978147600733805,
2.92774812072088E-17));
#121706=DIRECTION('ref_axis',(0.978147600733805,-0.207911690817763,-1.90483965589786E-31));
#121707=DIRECTION('center_axis',(-0.180084698747701,-0.8470874009056,-0.500012436349282));
#121708=DIRECTION('ref_axis',(0.102990311613069,0.489291521296384,-0.866017784402441));
#121709=DIRECTION('center_axis',(0.110177549147566,0.518344615107822,0.848044673146739));
#121710=DIRECTION('ref_axis',(1.88294772218094E-15,-0.853239260760981,0.521519667794088));
#121711=DIRECTION('center_axis',(0.103956877071345,0.489078702597146,0.866022511471536));
#121712=DIRECTION('ref_axis',(0.175675810167855,0.848020052664948,-0.500000000000007));
#121713=DIRECTION('center_axis',(-0.103956889752265,-0.489078713616244,
-0.866022503726384));
#121714=DIRECTION('ref_axis',(-5.684684706523E-16,0.870740345484775,-0.49174307391671));
#121715=DIRECTION('center_axis',(0.110177517566025,0.518344588176875,0.848044693710617));
#121716=DIRECTION('ref_axis',(0.171882402211048,0.830446875606581,-0.529919264233172));
#121717=DIRECTION('center_axis',(0.110177535564884,0.518344551206558,0.848044713969329));
#121718=DIRECTION('ref_axis',(1.68081909147871E-15,-0.853239300541055,0.521519602711357));
#121719=DIRECTION('center_axis',(-0.207911690817757,-0.978147600733806,
-2.83991567709928E-15));
#121720=DIRECTION('ref_axis',(0.978147600733806,-0.207911690817757,9.97553654791534E-32));
#121721=DIRECTION('center_axis',(0.207911690817754,0.978147600733807,0.));
#121722=DIRECTION('ref_axis',(-0.978147600733807,0.207911690817754,0.));
#121723=DIRECTION('center_axis',(-0.207911690817763,-0.978147600733805,
2.92774812072088E-17));
#121724=DIRECTION('ref_axis',(0.978147600733805,-0.207911690817763,-1.90483965589786E-31));
#121725=DIRECTION('center_axis',(-0.207911690817757,-0.978147600733806,
-1.98794097396939E-14));
#121726=DIRECTION('ref_axis',(0.978147600733806,-0.207911690817757,1.55832197481668E-31));
#121727=DIRECTION('center_axis',(-0.207911690817763,-0.978147600733805,
2.92774812072088E-17));
#121728=DIRECTION('ref_axis',(0.978147600733805,-0.207911690817763,-1.90483965589786E-31));
#121729=DIRECTION('center_axis',(0.18009299163103,0.847105178671961,-0.49997933020529));
#121730=DIRECTION('ref_axis',(0.104894406038834,0.488852904976947,0.866036951219381));
#121731=DIRECTION('center_axis',(-0.10395691792829,-0.489078846174021,0.866022425483278));
#121732=DIRECTION('ref_axis',(2.98952713487412E-15,-0.870740269393765,-0.491743208652721));
#121733=DIRECTION('center_axis',(-0.103956919794205,-0.48907885495245,0.86602242030175));
#121734=DIRECTION('ref_axis',(-0.978147600733542,0.207911690819,7.34320738951004E-13));
#121735=DIRECTION('center_axis',(0.154510046709505,0.47553302708606,0.86602250872376));
#121736=DIRECTION('ref_axis',(0.951056516296192,-0.309016994371752,-1.92322099198249E-12));
#121737=DIRECTION('center_axis',(0.267585776506576,0.823641557785139,0.500012436345979));
#121738=DIRECTION('ref_axis',(-0.15545353447118,-0.475234043094388,0.866017784404327));
#121739=DIRECTION('center_axis',(-0.154510049384291,-0.475533035318142,
-0.866022503726306));
#121740=DIRECTION('ref_axis',(-4.47004182862588E-15,0.876548788012434,-0.48131301897407));
#121741=DIRECTION('center_axis',(-0.309016994374972,-0.951056516295146,
0.));
#121742=DIRECTION('ref_axis',(0.951056516295146,-0.309016994374972,0.));
#121743=DIRECTION('center_axis',(0.309016994374951,0.951056516295152,-4.35148173242975E-17));
#121744=DIRECTION('ref_axis',(-0.951056516295152,0.309016994374951,-3.06907094049306E-33));
#121745=DIRECTION('center_axis',(0.309016994374964,0.951056516295148,0.));
#121746=DIRECTION('ref_axis',(-0.951056516295148,0.309016994374964,0.));
#121747=DIRECTION('center_axis',(0.309016994374951,0.951056516295152,-4.35148173242975E-17));
#121748=DIRECTION('ref_axis',(-0.951056516295152,0.309016994374951,4.2576019536567E-33));
#121749=DIRECTION('center_axis',(-0.309016994374922,-0.951056516295162,
0.));
#121750=DIRECTION('ref_axis',(0.951056516295162,-0.309016994374922,0.));
#121751=DIRECTION('center_axis',(0.163755587629901,0.503987876168977,-0.848045003637584));
#121752=DIRECTION('ref_axis',(-1.98200124493525E-15,0.859649462041493,0.510884333691857));
#121753=DIRECTION('center_axis',(-0.154510091261978,-0.475533164204395,
0.866022425483296));
#121754=DIRECTION('ref_axis',(5.93903874944703E-17,-0.876548714628845,-0.48131315261742));
#121755=DIRECTION('center_axis',(-0.163755599460449,-0.503987842609208,
0.848045021297493));
#121756=DIRECTION('ref_axis',(-0.266156470996902,-0.805199544424196,-0.529919264233282));
#121757=DIRECTION('center_axis',(0.163755570286413,0.50398782279121,-0.848045038708645));
#121758=DIRECTION('ref_axis',(-7.80935410721728E-16,0.8596494950837,0.51088427809274));
#121759=DIRECTION('center_axis',(-0.154510105543908,-0.47553317412871,0.866022417485762));
#121760=DIRECTION('ref_axis',(-0.271938812465217,-0.822222161143212,-0.499999999999993));
#121761=DIRECTION('center_axis',(-0.267587483539972,-0.823661100222839,
0.499979330205208));
#121762=DIRECTION('ref_axis',(-0.153585232132033,-0.475806237447057,-0.866036951219418));
#121763=DIRECTION('center_axis',(-0.950981553003154,0.309247612517397,0.));
#121764=DIRECTION('ref_axis',(-0.309247612517397,-0.950981553003154,0.));
#121765=DIRECTION('center_axis',(0.309016994374951,0.951056516295152,-4.35148173242975E-17));
#121766=DIRECTION('ref_axis',(-0.951056516295152,0.309016994374951,-3.06907094049306E-33));
#121767=DIRECTION('center_axis',(-0.309016994374972,-0.951056516295146,
0.));
#121768=DIRECTION('ref_axis',(0.951056516295146,-0.309016994374972,0.));
#121769=DIRECTION('center_axis',(-1.84331724214208E-16,-1.33924836902177E-16,
-1.));
#121770=DIRECTION('ref_axis',(-1.,-4.69758072753777E-33,2.25664243350207E-16));
#121771=DIRECTION('center_axis',(-0.951131423661017,0.308786358060986,0.));
#121772=DIRECTION('ref_axis',(-0.308786358060986,-0.951131423661017,0.));
#121773=DIRECTION('center_axis',(-0.163755730877694,-0.503988317040576,
-0.848044713969329));
#121774=DIRECTION('ref_axis',(1.26972035331881E-15,0.859649189130472,-0.510884792910615));
#121775=DIRECTION('center_axis',(-0.163755570286353,-0.503987822791173,
0.848045038708679));
#121776=DIRECTION('ref_axis',(-2.66055794635823E-15,-0.859649495083725,
-0.510884278092698));
#121777=DIRECTION('center_axis',(-0.163755716978191,-0.503988355849649,
-0.848044693589274));
#121778=DIRECTION('ref_axis',(0.266368911012766,0.805129291878272,-0.529919264233208));
#121779=DIRECTION('center_axis',(-0.163755751065448,-0.503988379172006,
-0.848044673146743));
#121780=DIRECTION('ref_axis',(-1.29103448395309E-15,0.859649150669466,-0.510884857627691));
#121781=DIRECTION('center_axis',(0.163755599580733,0.503987842736587,-0.848045021198566));
#121782=DIRECTION('ref_axis',(-0.257959309143581,-0.807862963763467,-0.529919264233216));
#121783=DIRECTION('center_axis',(-0.163755587629911,-0.503987876169007,
0.848045003637564));
#121784=DIRECTION('ref_axis',(1.65328349054603E-16,-0.859649462041474,-0.510884333691888));
#121785=DIRECTION('center_axis',(-0.950976702550718,0.309262527968978,9.08207363789492E-15));
#121786=DIRECTION('ref_axis',(-0.309262527968978,-0.950976702550718,-1.94816382726432E-29));
#121787=DIRECTION('center_axis',(-0.309016994374964,-0.951056516295148,
0.));
#121788=DIRECTION('ref_axis',(0.951056516295148,-0.309016994374964,0.));
#121789=DIRECTION('center_axis',(-1.84331724214208E-16,-1.33924836902177E-16,
-1.));
#121790=DIRECTION('ref_axis',(-1.,-6.6676823436159E-33,2.40228573745067E-16));
#121791=DIRECTION('center_axis',(-0.951136266645025,0.308771440182806,0.));
#121792=DIRECTION('ref_axis',(-0.308771440182806,-0.951136266645025,0.));
#121793=DIRECTION('center_axis',(-0.309016994374951,-0.951056516295152,
4.35148173242975E-17));
#121794=DIRECTION('ref_axis',(0.951056516295152,-0.309016994374951,3.88645736880897E-31));
#121795=DIRECTION('center_axis',(-0.267642920194759,-0.823622990673457,
-0.50001243634907));
#121796=DIRECTION('ref_axis',(0.153571010716792,0.475845712144077,-0.86601778440256));
#121797=DIRECTION('center_axis',(0.163755751065493,0.503988379172008,0.848044673146732));
#121798=DIRECTION('ref_axis',(-5.05660704346617E-15,-0.859649150669462,
0.510884857627698));
#121799=DIRECTION('center_axis',(0.154510035620874,0.475533025684823,0.86602251147154));
#121800=DIRECTION('ref_axis',(0.26335567263134,0.825011387614054,-0.500000000000027));
#121801=DIRECTION('center_axis',(-0.154510049384261,-0.475533035318047,
-0.866022503726363));
#121802=DIRECTION('ref_axis',(1.38257175086461E-15,0.876548788012488,-0.481313018973972));
#121803=DIRECTION('center_axis',(0.163755716843087,0.503988355689364,0.848044693710619));
#121804=DIRECTION('ref_axis',(0.257746148192743,0.80793099735453,-0.52991926423326));
#121805=DIRECTION('center_axis',(0.163755730877767,0.50398831704056,0.848044713969324));
#121806=DIRECTION('ref_axis',(-3.08584552958091E-15,-0.859649189130477,
0.510884792910606));
#121807=DIRECTION('center_axis',(-0.309016994374964,-0.951056516295148,
0.));
#121808=DIRECTION('ref_axis',(0.951056516295148,-0.309016994374964,0.));
#121809=DIRECTION('center_axis',(0.309016994374964,0.951056516295148,0.));
#121810=DIRECTION('ref_axis',(-0.951056516295148,0.309016994374964,0.));
#121811=DIRECTION('center_axis',(-0.309016994374951,-0.951056516295152,
4.35148173242975E-17));
#121812=DIRECTION('ref_axis',(0.951056516295152,-0.309016994374951,3.88645736880897E-31));
#121813=DIRECTION('center_axis',(-0.309016994374964,-0.951056516295148,
-6.88465858398752E-14));
#121814=DIRECTION('ref_axis',(0.951056516295148,-0.309016994374964,5.78888311337089E-28));
#121815=DIRECTION('center_axis',(-0.309016994374951,-0.951056516295152,
4.35148173242975E-17));
#121816=DIRECTION('ref_axis',(0.951056516295152,-0.309016994374951,3.88645736880897E-31));
#121817=DIRECTION('center_axis',(0.267653025931577,0.823639804208476,-0.499979330205854));
#121818=DIRECTION('ref_axis',(0.155418826432177,0.475210466544724,0.866036951219052));
#121819=DIRECTION('center_axis',(-0.154510091261975,-0.475533164204399,
0.866022425483295));
#121820=DIRECTION('ref_axis',(8.01177925627987E-16,-0.876548714628843,-0.481313152617424));
#121821=DIRECTION('center_axis',(-0.154510094034388,-0.475533172737027,
0.86602242030339));
#121822=DIRECTION('ref_axis',(-0.951056516296656,0.309016994370322,-2.79741233884318E-12));
#121823=DIRECTION('center_axis',(0.203370361062807,0.456777309669184,0.866022508721665));
#121824=DIRECTION('ref_axis',(0.913545457643418,-0.406736643073965,-1.18890024959013E-12));
#121825=DIRECTION('center_axis',(0.352213899941551,0.791159233141064,0.500012436348945));
#121826=DIRECTION('ref_axis',(-0.204277427942415,-0.456381342225541,0.866017784402633));
#121827=DIRECTION('center_axis',(-0.203370364581912,-0.456777317573273,
-0.86602250372631));
#121828=DIRECTION('ref_axis',(5.88898682911472E-15,0.884507036382098,-0.466526850878444));
#121829=DIRECTION('center_axis',(-0.406736643075807,-0.913545457642598,
0.));
#121830=DIRECTION('ref_axis',(0.913545457642598,-0.406736643075807,0.));
#121831=DIRECTION('center_axis',(0.406736643075804,0.913545457642599,-5.72753959967203E-17));
#121832=DIRECTION('ref_axis',(-0.913545457642599,0.406736643075804,-3.21579896619707E-33));
#121833=DIRECTION('center_axis',(0.406736643075807,0.913545457642598,0.));
#121834=DIRECTION('ref_axis',(-0.913545457642598,0.406736643075807,0.));
#121835=DIRECTION('center_axis',(0.406736643075804,0.913545457642599,-5.72753959967203E-17));
#121836=DIRECTION('ref_axis',(-0.913545457642599,0.406736643075804,-3.21579896619707E-33));
#121837=DIRECTION('center_axis',(-0.406736643075817,-0.913545457642594,
0.));
#121838=DIRECTION('ref_axis',(0.913545457642593,-0.406736643075817,0.));
#121839=DIRECTION('center_axis',(0.215539595588306,0.48410985792377,-0.848045003637576));
#121840=DIRECTION('ref_axis',(5.65310087418454E-16,0.868458021515995,0.495762710240013));
#121841=DIRECTION('center_axis',(-0.203370419702479,-0.456777441376134,
0.866022425483261));
#121842=DIRECTION('ref_axis',(-3.15644426060647E-15,-0.884506966812025,
-0.466526982779122));
#121843=DIRECTION('center_axis',(-0.21553960384998,-0.484109823309468,0.848045021297495));
#121844=DIRECTION('ref_axis',(-0.348864709042233,-0.772967650150662,-0.529919264233186));
#121845=DIRECTION('center_axis',(0.215539572760321,0.484109806651276,-0.848045038708654));
#121846=DIRECTION('ref_axis',(1.88184919665141E-15,0.868458052949964,0.495762655175193));
#121847=DIRECTION('center_axis',(-0.20337043494672,-0.456777449751744,0.866022417485757));
#121848=DIRECTION('ref_axis',(-0.356394722165886,-0.789292595944163,-0.500000000000026));
#121849=DIRECTION('center_axis',(-0.352217640366916,-0.791178490090378,
0.499979330205431));
#121850=DIRECTION('ref_axis',(-0.202479170969598,-0.457145692800741,-0.866036951219285));
#121851=DIRECTION('center_axis',(-0.913446798847324,0.406958162070226,0.));
#121852=DIRECTION('ref_axis',(-0.406958162070226,-0.913446798847324,0.));
#121853=DIRECTION('center_axis',(0.406736643075804,0.913545457642599,-5.72753959967203E-17));
#121854=DIRECTION('ref_axis',(-0.913545457642599,0.406736643075804,-3.21579896619707E-33));
#121855=DIRECTION('center_axis',(-0.406736643075817,-0.913545457642594,
0.));
#121856=DIRECTION('ref_axis',(0.913545457642593,-0.406736643075817,0.));
#121857=DIRECTION('center_axis',(-1.98092302886631E-16,-1.28642645648559E-16,
-1.));
#121858=DIRECTION('ref_axis',(-1.,-2.74025542439703E-33,2.25664243350207E-16));
#121859=DIRECTION('center_axis',(-0.913644062717546,0.406515100163544,0.));
#121860=DIRECTION('ref_axis',(-0.406515100163544,-0.913644062717546,0.));
#121861=DIRECTION('center_axis',(-0.21553978413504,-0.484110281406731,-0.848044713969326));
#121862=DIRECTION('ref_axis',(-4.09518441222106E-16,0.868457761888281,-0.495763165045567));
#121863=DIRECTION('center_axis',(-0.215539572760312,-0.484109806651254,
0.848045038708669));
#121864=DIRECTION('ref_axis',(2.33490112882762E-15,-0.868458052949978,-0.495762655175168));
#121865=DIRECTION('center_axis',(-0.215539774370682,-0.484110321455004,
-0.848044693589299));
#121866=DIRECTION('ref_axis',(0.349068641869932,0.772875576440141,-0.529919264233148));
#121867=DIRECTION('center_axis',(-0.215539810706662,-0.484110341087621,
-0.848044673146742));
#121868=DIRECTION('ref_axis',(2.48178269179927E-15,0.868457725299266,-0.495763229140711));
#121869=DIRECTION('center_axis',(0.215539603972856,0.484109823428023,-0.848045021198588));
#121870=DIRECTION('ref_axis',(-0.340990855181776,-0.776473315753338,-0.529919264233163));
#121871=DIRECTION('center_axis',(-0.215539595588304,-0.484109857923765,
0.84804500363758));
#121872=DIRECTION('ref_axis',(-1.76895097386485E-15,-0.868458021515998,
-0.495762710240009));
#121873=DIRECTION('center_axis',(-0.913440415876946,0.406972488803054,2.22357395402643E-14));
#121874=DIRECTION('ref_axis',(-0.406972488803054,-0.913440415876946,1.79710587910138E-28));
#121875=DIRECTION('center_axis',(-0.406736643075807,-0.913545457642598,
-1.11114268233636E-14));
#121876=DIRECTION('ref_axis',(0.913545457642598,-0.406736643075807,-1.88066567154315E-32));
#121877=DIRECTION('center_axis',(-1.98092302886631E-16,-1.28642645648559E-16,
-1.));
#121878=DIRECTION('ref_axis',(-1.,-4.68821414785493E-33,2.40228573745067E-16));
#121879=DIRECTION('center_axis',(-0.913650438514062,0.40650077023674,0.));
#121880=DIRECTION('ref_axis',(-0.40650077023674,-0.913650438514061,0.));
#121881=DIRECTION('center_axis',(-0.406736643075804,-0.913545457642599,
5.72753959967203E-17));
#121882=DIRECTION('ref_axis',(0.913545457642599,-0.406736643075804,-1.56826318575927E-31));
#121883=DIRECTION('center_axis',(-0.352268789800919,-0.791134794602218,
-0.500012436347239));
#121884=DIRECTION('ref_axis',(0.202469153662353,0.457186437804045,-0.866017784403588));
#121885=DIRECTION('center_axis',(0.215539810706706,0.484110341087606,0.848044673146739));
#121886=DIRECTION('ref_axis',(-5.01178427115621E-15,-0.868457725299272,
0.495763229140701));
#121887=DIRECTION('center_axis',(0.20337034988946,0.45677730943028,0.86602251147154));
#121888=DIRECTION('ref_axis',(0.348150155232207,0.79296372515504,-0.500000000000032));
#121889=DIRECTION('center_axis',(-0.203370364581871,-0.45677731757318,-0.866022503726368));
#121890=DIRECTION('ref_axis',(3.74161672221887E-15,0.88450703638215,-0.466526850878345));
#121891=DIRECTION('center_axis',(0.215539774220846,0.484110321309208,0.84804469371061));
#121892=DIRECTION('ref_axis',(0.340785973393292,0.776563258036921,-0.529919264233212));
#121893=DIRECTION('center_axis',(0.215539784135144,0.484110281406688,0.848044713969324));
#121894=DIRECTION('ref_axis',(-1.82583604731993E-15,-0.868457761888299,
0.495763165045535));
#121895=DIRECTION('center_axis',(-0.406736643075807,-0.913545457642598,
0.));
#121896=DIRECTION('ref_axis',(0.913545457642598,-0.406736643075807,0.));
#121897=DIRECTION('center_axis',(0.406736643075807,0.913545457642598,0.));
#121898=DIRECTION('ref_axis',(-0.913545457642598,0.406736643075807,0.));
#121899=DIRECTION('center_axis',(-0.406736643075804,-0.913545457642599,
5.72753959967203E-17));
#121900=DIRECTION('ref_axis',(0.913545457642599,-0.406736643075804,-1.56826318575927E-31));
#121901=DIRECTION('center_axis',(-0.406736643075807,-0.913545457642598,
2.22228536467272E-14));
#121902=DIRECTION('ref_axis',(0.913545457642598,-0.406736643075807,3.7613313430863E-32));
#121903=DIRECTION('center_axis',(-0.406736643075804,-0.913545457642599,
5.72753959967203E-17));
#121904=DIRECTION('ref_axis',(0.913545457642599,-0.406736643075804,-1.56826318575927E-31));
#121905=DIRECTION('center_axis',(0.352280597671145,0.791150459692763,-0.499979330205151));
#121906=DIRECTION('ref_axis',(0.204240445639906,0.456361522794511,0.866036951219454));
#121907=DIRECTION('center_axis',(-0.203370419702479,-0.456777441376094,
0.866022425483282));
#121908=DIRECTION('ref_axis',(-2.88067167725014E-15,-0.884506966812047,
-0.466526982779081));
#121909=DIRECTION('center_axis',(-0.203370423352518,-0.456777449574212,
0.866022420302094));
#121910=DIRECTION('ref_axis',(-0.913545457642604,0.406736643075794,0.));
#121911=DIRECTION('center_axis',(0.250002507181115,0.433017044457297,0.866022508721698));
#121912=DIRECTION('ref_axis',(0.86602540378529,-0.499999999998525,-9.79094323187051E-13));
#121913=DIRECTION('center_axis',(0.432983094184821,0.750008802378917,0.500012436349618));
#121914=DIRECTION('ref_axis',(-0.250863215193005,-0.432528431853988,0.866017784402236));
#121915=DIRECTION('center_axis',(-0.250002511507198,-0.433017051950279,
-0.866022503726308));
#121916=DIRECTION('ref_axis',(-6.20218011248958E-16,0.894424794863783,-0.447218387740127));
#121917=DIRECTION('center_axis',(-0.499999999999998,-0.86602540378444,-6.09762352041363E-14));
#121918=DIRECTION('ref_axis',(0.86602540378444,-0.499999999999998,8.3104781865219E-28));
#121919=DIRECTION('center_axis',(0.500000000000004,0.866025403784436,-7.04084534449558E-17));
#121920=DIRECTION('ref_axis',(-0.866025403784436,0.500000000000004,-7.94037779396281E-33));
#121921=DIRECTION('center_axis',(0.50000000000001,0.866025403784433,0.));
#121922=DIRECTION('ref_axis',(-0.866025403784433,0.50000000000001,0.));
#121923=DIRECTION('center_axis',(0.500000000000004,0.866025403784436,-7.04084534449558E-17));
#121924=DIRECTION('ref_axis',(-0.866025403784436,0.500000000000004,-7.94037779396281E-33));
#121925=DIRECTION('center_axis',(-0.50000000000001,-0.866025403784433,0.));
#121926=DIRECTION('ref_axis',(0.866025403784433,-0.50000000000001,0.));
#121927=DIRECTION('center_axis',(0.264962106632886,0.458927830768643,-0.848045003637573));
#121928=DIRECTION('ref_axis',(3.30353726242757E-15,0.879478602053321,0.4759384293481));
#121929=DIRECTION('center_axis',(-0.250002579266717,-0.433017169313223,
0.866022425483286));
#121930=DIRECTION('ref_axis',(-6.14028948685692E-15,-0.894424730216413,
-0.447218517033114));
#121931=DIRECTION('center_axis',(-0.264962111224684,-0.45892779548412,0.84804502129748));
#121932=DIRECTION('ref_axis',(-0.427750712264732,-0.732266960576195,-0.529919264233257));
#121933=DIRECTION('center_axis',(0.264962078570521,0.458927782163201,-0.848045038708649));
#121934=DIRECTION('ref_axis',(2.043795734415E-15,0.879478631391252,0.475938375135027));
#121935=DIRECTION('center_axis',(-0.250002595295631,-0.433017176053763,
0.866022417485756));
#121936=DIRECTION('ref_axis',(-0.43694589671013,-0.747715375893923,-0.499999999999991));
#121937=DIRECTION('center_axis',(-0.432988827019556,-0.750027562855828,
0.499979330205536));
#121938=DIRECTION('ref_axis',(-0.249154705644099,-0.433476564278061,-0.866036951219225));
#121939=DIRECTION('center_axis',(-0.865904130412325,0.500209992837883,0.));
#121940=DIRECTION('ref_axis',(-0.500209992837883,-0.865904130412325,0.));
#121941=DIRECTION('center_axis',(0.500000000000004,0.866025403784436,-7.04084534449558E-17));
#121942=DIRECTION('ref_axis',(-0.866025403784436,0.500000000000004,-7.94037779396281E-33));
#121943=DIRECTION('center_axis',(-0.500000000000022,-0.866025403784426,
0.));
#121944=DIRECTION('ref_axis',(0.866025403784426,-0.500000000000022,0.));
#121945=DIRECTION('center_axis',(-2.11225360334866E-16,-1.2195101864901E-16,
-1.));
#121946=DIRECTION('ref_axis',(-1.,-1.17439518188444E-33,2.25664243350207E-16));
#121947=DIRECTION('center_axis',(-0.866146626230631,0.499789977759954,0.));
#121948=DIRECTION('ref_axis',(-0.499789977759954,-0.866146626230631,0.));
#121949=DIRECTION('center_axis',(-0.264962338412801,-0.458928232223203,
-0.84804471396932));
#121950=DIRECTION('ref_axis',(1.63607178079679E-15,0.879478359737744,-0.475938877118698));
#121951=DIRECTION('center_axis',(-0.264962078570535,-0.458927782163211,
0.848045038708639));
#121952=DIRECTION('ref_axis',(1.55530095974517E-15,-0.879478631391246,-0.475938375135039));
#121953=DIRECTION('center_axis',(-0.264962332884843,-0.458928273074652,
-0.848044693589282));
#121954=DIRECTION('ref_axis',(0.42794390361672,0.732154074462357,-0.529919264233198));
#121955=DIRECTION('center_axis',(-0.264962371077225,-0.458928288799661,
-0.848044673146733));
#121956=DIRECTION('ref_axis',(2.91201203045915E-15,0.879478325588505,-0.475938940222419));
#121957=DIRECTION('center_axis',(0.264962111365172,0.458927795585784,-0.84804502119857));
#121958=DIRECTION('ref_axis',(-0.420286434086469,-0.736576463591759,-0.529919264233277));
#121959=DIRECTION('center_axis',(-0.264962106632899,-0.458927830768652,
0.848045003637564));
#121960=DIRECTION('ref_axis',(-1.62952198067E-16,-0.879478602053315,-0.47593842934811));
#121961=DIRECTION('center_axis',(-0.865896284857136,0.500223573885327,3.67572504896101E-15));
#121962=DIRECTION('ref_axis',(-0.500223573885327,-0.865896284857136,-1.1847470281813E-29));
#121963=DIRECTION('center_axis',(-0.50000000000001,-0.866025403784433,1.36592399683214E-14));
#121964=DIRECTION('ref_axis',(0.866025403784433,-0.50000000000001,-3.78074180857848E-32));
#121965=DIRECTION('center_axis',(-2.11225360334866E-16,-1.2195101864901E-16,
-1.));
#121966=DIRECTION('ref_axis',(-1.,-2.81292848871296E-33,2.40228573745067E-16));
#121967=DIRECTION('center_axis',(-0.866154464985103,0.499776392786184,-2.7306262718275E-14));
#121968=DIRECTION('ref_axis',(-0.499776392786184,-0.866154464985103,-3.39882034587859E-28));
#121969=DIRECTION('center_axis',(-0.500000000000004,-0.866025403784436,
7.04084534449558E-17));
#121970=DIRECTION('ref_axis',(0.866025403784436,-0.500000000000004,-4.66754835686058E-31));
#121971=DIRECTION('center_axis',(-0.433035128829375,-0.749978760163243,
-0.500012436349069));
#121972=DIRECTION('ref_axis',(0.249149002240728,0.433518133162794,-0.866017784402547));
#121973=DIRECTION('center_axis',(0.264962371077208,0.45892828879966,0.848044673146739));
#121974=DIRECTION('ref_axis',(-3.94378445652297E-15,-0.879478325588507,
0.475938940222416));
#121975=DIRECTION('center_axis',(0.250002496041659,0.433017045389097,0.866022511471519));
#121976=DIRECTION('ref_axis',(0.429130231859143,0.752228186193846,-0.500000000000034));
#121977=DIRECTION('center_axis',(-0.250002511507148,-0.433017051950192,
-0.866022503726366));
#121978=DIRECTION('ref_axis',(-4.43899159512102E-15,0.894424794863831,-0.447218387740031));
#121979=DIRECTION('center_axis',(0.264962332718263,0.458928272946614,0.848044693710617));
#121980=DIRECTION('ref_axis',(0.420092076154909,0.736687329161024,-0.529919264233199));
#121981=DIRECTION('center_axis',(0.264962338412815,0.458928232223191,0.848044713969322));
#121982=DIRECTION('ref_axis',(-4.71779924553047E-15,-0.879478359737749,
0.475938877118689));
#121983=DIRECTION('center_axis',(-0.50000000000001,-0.866025403784433,-4.73169952358149E-14));
#121984=DIRECTION('ref_axis',(0.866025403784433,-0.50000000000001,9.25800991341574E-31));
#121985=DIRECTION('center_axis',(0.50000000000001,0.866025403784433,0.));
#121986=DIRECTION('ref_axis',(-0.866025403784433,0.50000000000001,0.));
#121987=DIRECTION('center_axis',(-0.500000000000004,-0.866025403784436,
7.04084534449558E-17));
#121988=DIRECTION('ref_axis',(0.866025403784436,-0.500000000000004,-4.66754835686058E-31));
#121989=DIRECTION('center_axis',(-0.50000000000001,-0.866025403784433,-1.35611710376594E-13));
#121990=DIRECTION('ref_axis',(0.866025403784433,-0.50000000000001,3.75412068987699E-30));
#121991=DIRECTION('center_axis',(-0.500000000000004,-0.866025403784436,
7.04084534449558E-17));
#121992=DIRECTION('ref_axis',(0.866025403784436,-0.500000000000004,-4.66754835686058E-31));
#121993=DIRECTION('center_axis',(0.433048509461931,0.749993105181681,-0.4999793302055));
#121994=DIRECTION('ref_axis',(0.250824363779151,0.432512586704298,0.866036951219254));
#121995=DIRECTION('center_axis',(-0.250002579266721,-0.433017169313215,
0.866022425483288));
#121996=DIRECTION('ref_axis',(3.65468156859272E-15,-0.894424730216417,-0.447218517033104));
#121997=DIRECTION('center_axis',(-0.250002583753713,-0.433017177084928,
0.866022420302078));
#121998=DIRECTION('ref_axis',(-0.86602540378536,0.499999999998404,-1.08399728131085E-12));
#121999=DIRECTION('center_axis',(0.293895573516567,0.404512553894631,0.866022508719613));
#122000=DIRECTION('ref_axis',(0.809016994374147,-0.587785252293575,7.34320742400955E-13));
#122001=DIRECTION('center_axis',(0.509008435042963,0.700641118228318,0.500012436348224));
#122002=DIRECTION('ref_axis',(-0.294700492539324,-0.403936649481947,0.866017784403056));
#122003=DIRECTION('center_axis',(-0.293895578600006,-0.404512560891467,
-0.866022503726315));
#122004=DIRECTION('ref_axis',(-5.69513563873506E-15,0.906035256115484,-0.423202214875761));
#122005=DIRECTION('center_axis',(-0.58778525229247,-0.80901699437495,0.));
#122006=DIRECTION('ref_axis',(0.80901699437495,-0.58778525229247,0.));
#122007=DIRECTION('center_axis',(0.587785252292477,0.809016994374945,-8.27701011433323E-17));
#122008=DIRECTION('ref_axis',(-0.809016994374945,0.587785252292477,1.49515186639062E-33));
#122009=DIRECTION('center_axis',(0.587785252292496,0.809016994374931,0.));
#122010=DIRECTION('ref_axis',(-0.809016994374931,0.587785252292496,0.));
#122011=DIRECTION('center_axis',(0.587785252292477,0.809016994374945,-8.27701011433323E-17));
#122012=DIRECTION('ref_axis',(-0.809016994374945,0.587785252292477,1.49515186639062E-33));
#122013=DIRECTION('center_axis',(-0.58778525229247,-0.80901699437495,0.));
#122014=DIRECTION('ref_axis',(0.80901699437495,-0.58778525229247,0.));
#122015=DIRECTION('center_axis',(0.311481637390311,0.428717694262756,-0.848045003637588));
#122016=DIRECTION('ref_axis',(-6.50621339553239E-15,0.892442058026273,0.451162025292277));
#122017=DIRECTION('center_axis',(-0.293895658256084,-0.404512670528678,
0.866022425483301));
#122018=DIRECTION('ref_axis',(2.74693569375712E-15,-0.906035197473498,-0.423202340422592));
#122019=DIRECTION('center_axis',(-0.311481638270574,-0.42871765869024,0.848045021297477));
#122020=DIRECTION('ref_axis',(-0.501950189192533,-0.683543400936663,-0.52991926423326));
#122021=DIRECTION('center_axis',(0.311481604401037,0.428717648856917,-0.848045038708649));
#122022=DIRECTION('ref_axis',(7.95334372440912E-15,0.892442084777736,0.451161972375297));
#122023=DIRECTION('center_axis',(-0.293895674908046,-0.404512675552269,
0.866022417485765));
#122024=DIRECTION('ref_axis',(-0.512709800570221,-0.697946029718086,-0.500000000000004));
#122025=DIRECTION('center_axis',(-0.509016097474224,-0.7006591766899,0.499979330205102));
#122026=DIRECTION('ref_axis',(-0.293100449236653,-0.405058175796668,-0.866036951219489));
#122027=DIRECTION('center_axis',(-0.808874435122379,0.587981418248444,0.));
#122028=DIRECTION('ref_axis',(-0.587981418248444,-0.808874435122379,0.));
#122029=DIRECTION('center_axis',(0.587785252292477,0.809016994374945,-8.27701011433323E-17));
#122030=DIRECTION('ref_axis',(-0.809016994374945,0.587785252292477,1.49515186639062E-33));
#122031=DIRECTION('center_axis',(-0.58778525229247,-0.80901699437495,0.));
#122032=DIRECTION('ref_axis',(0.80901699437495,-0.58778525229247,0.));
#122033=DIRECTION('center_axis',(-2.23587008033243E-16,-1.13923270769252E-16,
-1.));
#122034=DIRECTION('ref_axis',(-1.,3.91465060628147E-34,2.25664243350207E-16));
#122035=DIRECTION('center_axis',(-0.809159506053914,0.587589051772227,0.));
#122036=DIRECTION('ref_axis',(-0.587589051772227,-0.809159506053914,0.));
#122037=DIRECTION('center_axis',(-0.311481909863919,-0.428718069290544,
-0.848044713969325));
#122038=DIRECTION('ref_axis',(5.77422614531214E-15,0.892441837073393,-0.451162462358149));
#122039=DIRECTION('center_axis',(-0.311481604401053,-0.428717648856938,
0.848045038708632));
#122040=DIRECTION('ref_axis',(2.51748144391242E-16,-0.892442084777725,-0.451161972375319));
#122041=DIRECTION('center_axis',(-0.311481908632573,-0.428718110498838,
-0.848044693589268));
#122042=DIRECTION('ref_axis',(0.502130522422689,0.683410939220382,-0.529919264233177));
#122043=DIRECTION('center_axis',(-0.31148194826326,-0.428718122142703,-0.848044673146738));
#122044=DIRECTION('ref_axis',(-5.37120173115187E-15,0.892441805934777,-0.451162523953258));
#122045=DIRECTION('center_axis',(0.31148163842248,0.428717658775535,-0.848045021198563));
#122046=DIRECTION('ref_axis',(-0.494977266821892,-0.688609525583308,-0.529919264233205));
#122047=DIRECTION('center_axis',(-0.311481637390301,-0.428717694262743,
0.848045003637598));
#122048=DIRECTION('ref_axis',(1.33996802632922E-15,-0.892442058026281,-0.451162025292263));
#122049=DIRECTION('center_axis',(-0.808865212939984,0.587994104813606,0.));
#122050=DIRECTION('ref_axis',(-0.587994104813606,-0.808865212939984,0.));
#122051=DIRECTION('center_axis',(-0.587785252292496,-0.809016994374931,
0.));
#122052=DIRECTION('ref_axis',(0.809016994374931,-0.587785252292496,0.));
#122053=DIRECTION('center_axis',(-2.23587008033243E-16,-1.13923270769252E-16,
-1.));
#122054=DIRECTION('ref_axis',(-1.,-1.25019043942798E-33,2.40228573745067E-16));
#122055=DIRECTION('center_axis',(-0.80916872188328,0.587576360591353,-3.2103386036122E-14));
#122056=DIRECTION('ref_axis',(-0.587576360591353,-0.809168721883279,4.76085920470349E-28));
#122057=DIRECTION('center_axis',(-0.587785252292477,-0.809016994374945,
8.27701011433323E-17));
#122058=DIRECTION('ref_axis',(0.809016994374945,-0.587785252292477,-5.76465719897875E-31));
#122059=DIRECTION('center_axis',(-0.509057044368004,-0.700605801485533,
-0.500012436349463));
#122060=DIRECTION('ref_axis',(0.293099122190527,0.405100113144951,-0.866017784402313));
#122061=DIRECTION('center_axis',(0.311481948263274,0.428718122142712,0.848044673146729));
#122062=DIRECTION('ref_axis',(-5.17619376781642E-15,-0.892441805934769,
0.451162523953273));
#122063=DIRECTION('center_axis',(0.293895562533816,0.404512555982461,0.866022511471537));
#122064=DIRECTION('ref_axis',(0.505408667886166,0.703251077799033,-0.500000000000029));
#122065=DIRECTION('center_axis',(-0.293895578599989,-0.404512560891416,
-0.866022503726345));
#122066=DIRECTION('ref_axis',(-2.21255256144257E-15,0.906035256115509,-0.423202214875706));
#122067=DIRECTION('center_axis',(0.311481908458004,0.428718110385629,0.848044693710618));
#122068=DIRECTION('ref_axis',(0.494795562235362,0.688740099737728,-0.5299192642332));
#122069=DIRECTION('center_axis',(0.311481909863932,0.428718069290522,0.848044713969331));
#122070=DIRECTION('ref_axis',(9.11251128025232E-15,-0.892441837073405,0.451162462358124));
#122071=DIRECTION('center_axis',(-0.587785252292496,-0.809016994374931,
-7.63170283020816E-14));
#122072=DIRECTION('ref_axis',(0.809016994374931,-0.587785252292496,-1.1810600377477E-30));
#122073=DIRECTION('center_axis',(0.587785252292496,0.809016994374931,0.));
#122074=DIRECTION('ref_axis',(-0.809016994374931,0.587785252292496,0.));
#122075=DIRECTION('center_axis',(-0.587785252292477,-0.809016994374945,
8.27701011433323E-17));
#122076=DIRECTION('ref_axis',(0.809016994374945,-0.587785252292477,-5.76465719897875E-31));
#122077=DIRECTION('center_axis',(-0.587785252292496,-0.809016994374931,
0.));
#122078=DIRECTION('ref_axis',(0.809016994374931,-0.587785252292496,0.));
#122079=DIRECTION('center_axis',(-0.587785252292477,-0.809016994374945,
8.27701011433323E-17));
#122080=DIRECTION('ref_axis',(0.809016994374945,-0.587785252292477,-5.76465719897875E-31));
#122081=DIRECTION('center_axis',(0.509071851162668,0.700618669263909,-0.499979330205442));
#122082=DIRECTION('ref_axis',(0.294660197703196,0.403924952203149,0.866036951219287));
#122083=DIRECTION('center_axis',(-0.293895658256125,-0.404512670528681,
0.866022425483286));
#122084=DIRECTION('ref_axis',(5.42521881944202E-15,-0.906035197473494,-0.4232023404226));
#122085=DIRECTION('center_axis',(-0.293895663530527,-0.404512677788301,
0.866022420302436));
#122086=DIRECTION('ref_axis',(-0.809016994372353,0.587785252296044,2.55263875924096E-12));
#122087=DIRECTION('center_axis',(0.334568658441521,0.371576139134707,0.866022508722715));
#122088=DIRECTION('ref_axis',(0.743144825480459,-0.669130606355454,-2.65754173435105E-12));
#122089=DIRECTION('center_axis',(0.579456972966894,0.643597063368936,0.500012436348264));
#122090=DIRECTION('ref_axis',(-0.335308969645359,-0.370919252631962,0.866017784403019));
#122091=DIRECTION('center_axis',(-0.334568664232084,-0.371576145565852,
-0.866022503726309));
#122092=DIRECTION('ref_axis',(-7.22273520455772E-15,0.918982183096513,-0.394299058014557));
#122093=DIRECTION('center_axis',(-0.669130606358875,-0.743144825477379,
0.));
#122094=DIRECTION('ref_axis',(0.743144825477379,-0.669130606358875,0.));
#122095=DIRECTION('center_axis',(0.669130606358862,0.743144825477391,-9.42249022928252E-17));
#122096=DIRECTION('ref_axis',(-0.743144825477391,0.669130606358862,5.64385269611616E-33));
#122097=DIRECTION('center_axis',(0.669130606358845,0.743144825477406,3.25153501695813E-14));
#122098=DIRECTION('ref_axis',(-0.743144825477406,0.669130606358845,-2.32720619691874E-30));
#122099=DIRECTION('center_axis',(0.669130606358862,0.743144825477391,-9.42249022928252E-17));
#122100=DIRECTION('ref_axis',(-0.743144825477391,0.669130606358862,5.64385269611616E-33));
#122101=DIRECTION('center_axis',(-0.669130606358872,-0.743144825477382,
0.));
#122102=DIRECTION('ref_axis',(0.743144825477382,-0.669130606358872,0.));
#122103=DIRECTION('center_axis',(0.354588510146763,0.393810436983647,-0.848045003637571));
#122104=DIRECTION('ref_axis',(2.71562606242776E-17,0.906978223357759,0.421177518814577));
#122105=DIRECTION('center_axis',(-0.334568754912021,-0.371576246276125,
0.866022425483293));
#122106=DIRECTION('ref_axis',(6.32948812453082E-15,-0.918982131463643,-0.394299178353873));
#122107=DIRECTION('center_axis',(-0.354588507312263,-0.393810401506322,
0.848045021297508));
#122108=DIRECTION('ref_axis',(-0.570650194832095,-0.627330796735366,-0.529919264233206));
#122109=DIRECTION('center_axis',(0.354588472592004,0.393810395274862,-0.848045038708633));
#122110=DIRECTION('ref_axis',(1.64363307278047E-15,0.906978247051285,0.421177467792116));
#122111=DIRECTION('center_axis',(-0.334568771992555,-0.371576249536343,
0.866022417485771));
#122112=DIRECTION('ref_axis',(-0.582856348570488,-0.640529840781128,-0.49999999999998));
#122113=DIRECTION('center_axis',(-0.579466481046732,-0.643614221961325,
0.499979330205196));
#122114=DIRECTION('ref_axis',(-0.333834922958285,-0.372201885185958,-0.866036951219435));
#122115=DIRECTION('center_axis',(-0.742982542253438,0.669310796197565,0.));
#122116=DIRECTION('ref_axis',(-0.669310796197565,-0.742982542253438,0.));
#122117=DIRECTION('center_axis',(0.669130606358862,0.743144825477391,-9.42249022928252E-17));
#122118=DIRECTION('ref_axis',(-0.743144825477391,0.669130606358862,5.64385269611616E-33));
#122119=DIRECTION('center_axis',(-0.669130606358869,-0.743144825477384,
0.));
#122120=DIRECTION('ref_axis',(0.743144825477384,-0.669130606358869,0.));
#122121=DIRECTION('center_axis',(-2.35041809182736E-16,-1.04647355694969E-16,
-1.));
#122122=DIRECTION('ref_axis',(-1.,1.56586024251259E-33,2.25664243350207E-16));
#122123=DIRECTION('center_axis',(-0.743307065001301,0.668950377172442,0.));
#122124=DIRECTION('ref_axis',(-0.668950377172442,-0.743307065001301,0.));
#122125=DIRECTION('center_axis',(-0.35458882032882,-0.393810781475684,-0.848044713969332));
#122126=DIRECTION('ref_axis',(2.88783290955208E-15,0.906978027661852,-0.421177940232649));
#122127=DIRECTION('center_axis',(-0.354588472592003,-0.393810395274861,
0.848045038708634));
#122128=DIRECTION('ref_axis',(-2.07668913976795E-15,-0.906978247051285,
-0.421177467792115));
#122129=DIRECTION('center_axis',(-0.35458882341487,-0.393810822584025,-0.848044693589289));
#122130=DIRECTION('ref_axis',(0.570815694127792,0.627180210730487,-0.529919264233212));
#122131=DIRECTION('center_axis',(-0.354588864042336,-0.393810830024532,
-0.848044673146736));
#122132=DIRECTION('ref_axis',(1.70751137071295E-15,0.906978000082644,-0.421177999622591));
#122133=DIRECTION('center_axis',(0.3545885074659,0.393810401581074,-0.848045021198556));
#122134=DIRECTION('ref_axis',(-0.564245025066716,-0.633098037496543,-0.529919264233229));
#122135=DIRECTION('center_axis',(-0.354588510146757,-0.393810436983641,
0.848045003637576));
#122136=DIRECTION('ref_axis',(4.72845601854126E-15,-0.906978223357763,-0.421177518814568));
#122137=DIRECTION('center_axis',(-0.742972044483925,0.669322449283883,0.));
#122138=DIRECTION('ref_axis',(-0.669322449283883,-0.742972044483925,0.));
#122139=DIRECTION('center_axis',(-0.669130606358845,-0.743144825477406,
0.));
#122140=DIRECTION('ref_axis',(0.743144825477406,-0.669130606358845,0.));
#122141=DIRECTION('center_axis',(-2.35041809182736E-16,-1.04647355694969E-16,
-1.));
#122142=DIRECTION('ref_axis',(-1.,0.,2.40228573745067E-16));
#122143=DIRECTION('center_axis',(-0.743317556935059,0.668938718831625,0.));
#122144=DIRECTION('ref_axis',(-0.668938718831625,-0.743317556935059,0.));
#122145=DIRECTION('center_axis',(-0.669130606358862,-0.743144825477391,
9.42249022928252E-17));
#122146=DIRECTION('ref_axis',(0.743144825477391,-0.669130606358862,-1.48947931215863E-30));
#122147=DIRECTION('center_axis',(-0.579501624400555,-0.643556859036987,
-0.500012436348903));
#122148=DIRECTION('ref_axis',(0.333837986843671,0.372243731496557,-0.866017784402655));
#122149=DIRECTION('center_axis',(0.354588864042412,0.393810830024454,0.848044673146741));
#122150=DIRECTION('ref_axis',(-1.10267543862293E-14,-0.906978000082675,
0.421177999622524));
#122151=DIRECTION('center_axis',(0.334568647739183,0.37157614236448,0.866022511471559));
#122152=DIRECTION('ref_axis',(0.576149740773813,0.64656900343761,-0.499999999999964));
#122153=DIRECTION('center_axis',(-0.334568664232057,-0.371576145565822,
-0.866022503726331));
#122154=DIRECTION('ref_axis',(4.82085454881383E-15,0.918982183096526,-0.394299058014526));
#122155=DIRECTION('center_axis',(0.354588823231024,0.393810822488337,0.848044693710595));
#122156=DIRECTION('ref_axis',(0.564077964596703,0.633246889649659,-0.529919264233216));
#122157=DIRECTION('center_axis',(0.354588820328813,0.393810781475714,0.848044713969321));
#122158=DIRECTION('ref_axis',(8.39746514209146E-15,-0.906978027661839,0.421177940232676));
#122159=DIRECTION('center_axis',(-0.669130606358845,-0.743144825477406,
3.65592620896146E-14));
#122160=DIRECTION('ref_axis',(0.743144825477406,-0.669130606358845,9.99649599890217E-31));
#122161=DIRECTION('center_axis',(0.669130606358875,0.743144825477379,0.));
#122162=DIRECTION('ref_axis',(-0.743144825477379,0.669130606358875,0.));
#122163=DIRECTION('center_axis',(-0.669130606358862,-0.743144825477391,
9.42249022928252E-17));
#122164=DIRECTION('ref_axis',(0.743144825477391,-0.669130606358862,-1.48947931215863E-30));
#122165=DIRECTION('center_axis',(-0.669130606358845,-0.743144825477406,
4.0439119200333E-15));
#122166=DIRECTION('ref_axis',(0.743144825477406,-0.669130606358845,-2.12202718326909E-31));
#122167=DIRECTION('center_axis',(-0.669130606358862,-0.743144825477391,
9.42249022928252E-17));
#122168=DIRECTION('ref_axis',(0.743144825477391,-0.669130606358862,-1.48947931215863E-30));
#122169=DIRECTION('center_axis',(0.579517695132025,0.643568108591859,-0.499979330205122));
#122170=DIRECTION('ref_axis',(0.335267672838056,0.37091183139964,0.866036951219472));
#122171=DIRECTION('center_axis',(-0.334568754912014,-0.371576246276117,
0.866022425483298));
#122172=DIRECTION('ref_axis',(3.2863782672971E-15,-0.918982131463647,-0.394299178353865));
#122173=DIRECTION('center_axis',(-0.334568760917623,-0.37157625294595,0.8660224203014));
#122174=DIRECTION('ref_axis',(-0.743144825474898,0.66913060636163,2.13302690841267E-12));
#122175=DIRECTION('center_axis',(0.371576139135906,0.334568658442567,0.866022508721797));
#122176=DIRECTION('ref_axis',(0.669130606361539,-0.743144825474981,-2.06309160956524E-12));
#122177=DIRECTION('center_axis',(0.643556859037152,0.579501624400958,0.500012436348223));
#122178=DIRECTION('ref_axis',(-0.37224373150869,-0.333837986829168,0.866017784403031));
#122179=DIRECTION('center_axis',(-0.371576145565853,-0.334568664232085,
-0.866022503726308));
#122180=DIRECTION('ref_axis',(-0.918982183096513,7.65889573873005E-15,0.394299058014558));
#122181=DIRECTION('center_axis',(-0.743144825477406,-0.669130606358845,
-3.65592620896146E-14));
#122182=DIRECTION('ref_axis',(0.669130606358845,-0.743144825477406,1.03271697859918E-30));
#122183=DIRECTION('center_axis',(0.743144825477398,0.669130606358854,-1.04647355694969E-16));
#122184=DIRECTION('ref_axis',(-0.669130606358854,0.743144825477398,-9.32318254549198E-33));
#122185=DIRECTION('center_axis',(0.743144825477406,0.669130606358845,0.));
#122186=DIRECTION('ref_axis',(-0.669130606358845,0.743144825477406,0.));
#122187=DIRECTION('center_axis',(0.743144825477398,0.669130606358854,-1.04647355694969E-16));
#122188=DIRECTION('ref_axis',(-0.669130606358854,0.743144825477398,-9.32318254549198E-33));
#122189=DIRECTION('center_axis',(-0.743144825477382,-0.669130606358872,
0.));
#122190=DIRECTION('ref_axis',(0.669130606358872,-0.743144825477382,0.));
#122191=DIRECTION('center_axis',(0.393810436983641,0.354588510146757,-0.848045003637576));
#122192=DIRECTION('ref_axis',(-0.906978223357763,4.7283308664863E-15,-0.421177518814568));
#122193=DIRECTION('center_axis',(-0.371576246276136,-0.334568754912019,
0.866022425483288));
#122194=DIRECTION('ref_axis',(0.918982131463639,-1.04034049828032E-14,0.394299178353883));
#122195=DIRECTION('center_axis',(-0.393810430453513,-0.354588475163147,
0.848045021297509));
#122196=DIRECTION('ref_axis',(-0.633098037500157,-0.564245025062705,-0.529919264233181));
#122197=DIRECTION('center_axis',(0.393810395274834,0.354588472591979,-0.848045038708656));
#122198=DIRECTION('ref_axis',(-0.906978247051303,9.86594956512546E-15,-0.421177467792077));
#122199=DIRECTION('center_axis',(-0.371576263603857,-0.334568756369017,
0.866022417485764));
#122200=DIRECTION('ref_axis',(-0.646617000434433,-0.576095872879835,-0.499999999999998));
#122201=DIRECTION('center_axis',(-0.6435681085917,-0.579517695132229,0.49997933020509));
#122202=DIRECTION('ref_axis',(-0.370911831392187,-0.335267672846279,-0.866036951219482));
#122203=DIRECTION('center_axis',(-0.668950377172403,0.743307065001336,0.));
#122204=DIRECTION('ref_axis',(-0.743307065001336,-0.668950377172402,0.));
#122205=DIRECTION('center_axis',(0.743144825477398,0.669130606358854,-1.04647355694969E-16));
#122206=DIRECTION('ref_axis',(-0.669130606358854,0.743144825477398,-9.32318254549198E-33));
#122207=DIRECTION('center_axis',(-0.743144825477382,-0.669130606358872,
0.));
#122208=DIRECTION('ref_axis',(0.669130606358872,-0.743144825477382,0.));
#122209=DIRECTION('center_axis',(-2.4546426258488E-16,-9.42249022928242E-17,
-1.));
#122210=DIRECTION('ref_axis',(-1.,2.34879036376888E-33,2.25664243350207E-16));
#122211=DIRECTION('center_axis',(-0.669310796197597,0.742982542253409,0.));
#122212=DIRECTION('ref_axis',(-0.742982542253409,-0.669310796197597,0.));
#122213=DIRECTION('center_axis',(-0.393810781475716,-0.35458882032887,-0.848044713969297));
#122214=DIRECTION('ref_axis',(-0.906978027661832,-3.75249855275816E-15,
0.421177940232692));
#122215=DIRECTION('center_axis',(-0.393810395274935,-0.354588472592007,
0.848045038708598));
#122216=DIRECTION('ref_axis',(0.90697824705125,-1.0449597276298E-14,0.42117746779219));
#122217=DIRECTION('center_axis',(-0.393810788842373,-0.35458886088878,-0.848044693589285));
#122218=DIRECTION('ref_axis',(0.633246889661538,0.564077964583415,-0.529919264233165));
#122219=DIRECTION('center_axis',(-0.393810830024481,-0.354588864042382,
-0.848044673146741));
#122220=DIRECTION('ref_axis',(-0.906978000082665,-2.2872769161124E-15,0.421177999622545));
#122221=DIRECTION('center_axis',(0.393810430611346,0.354588475224443,-0.848045021198586));
#122222=DIRECTION('ref_axis',(-0.627330796759002,-0.570650194806061,-0.52991926423326));
#122223=DIRECTION('center_axis',(-0.393810436983659,-0.354588510146774,
0.848045003637561));
#122224=DIRECTION('ref_axis',(0.906978223357753,-5.41285892759898E-15,0.42117751881459));
#122225=DIRECTION('center_axis',(-0.668938718831589,0.743317556935091,0.));
#122226=DIRECTION('ref_axis',(-0.743317556935091,-0.668938718831589,0.));
#122227=DIRECTION('center_axis',(-0.743144825477406,-0.669130606358845,
0.));
#122228=DIRECTION('ref_axis',(0.669130606358845,-0.743144825477406,0.));
#122229=DIRECTION('center_axis',(-2.4546426258488E-16,-9.42249022928242E-17,
-1.));
#122230=DIRECTION('ref_axis',(-1.,1.04182536618998E-33,2.40228573745067E-16));
#122231=DIRECTION('center_axis',(-0.669322449283883,0.742972044483925,0.));
#122232=DIRECTION('ref_axis',(-0.742972044483925,-0.669322449283883,0.));
#122233=DIRECTION('center_axis',(-0.743144825477398,-0.669130606358854,
1.04647355694969E-16));
#122234=DIRECTION('ref_axis',(0.669130606358854,-0.743144825477398,-1.33231393542051E-30));
#122235=DIRECTION('center_axis',(-0.643597063368147,-0.579456972967606,
-0.500012436348454));
#122236=DIRECTION('ref_axis',(0.370919252632461,0.335308969645089,-0.86601778440291));
#122237=DIRECTION('center_axis',(0.393810830024549,0.354588864042318,0.848044673146736));
#122238=DIRECTION('ref_axis',(0.906978000082638,-3.66139072703648E-15,-0.421177999622604));
#122239=DIRECTION('center_axis',(0.371576128828018,0.334568662772985,0.866022511471544));
#122240=DIRECTION('ref_axis',(0.640578396533018,0.582802983773409,-0.499999999999999));
#122241=DIRECTION('center_axis',(-0.371576145565821,-0.334568664232056,
-0.866022503726332));
#122242=DIRECTION('ref_axis',(-0.918982183096527,-5.2693457410403E-15,0.394299058014525));
#122243=DIRECTION('center_axis',(0.393810788647791,0.354588860814735,0.848044693710605));
#122244=DIRECTION('ref_axis',(0.627180210739902,0.570815694117418,-0.529919264233244));
#122245=DIRECTION('center_axis',(0.39381078147571,0.354588820328817,0.848044713969322));
#122246=DIRECTION('ref_axis',(0.906978027661841,-6.75609972193682E-15,-0.421177940232673));
#122247=DIRECTION('center_axis',(-0.743144825477406,-0.669130606358845,
0.));
#122248=DIRECTION('ref_axis',(0.669130606358845,-0.743144825477406,0.));
#122249=DIRECTION('center_axis',(0.743144825477406,0.669130606358845,0.));
#122250=DIRECTION('ref_axis',(-0.669130606358845,0.743144825477406,0.));
#122251=DIRECTION('center_axis',(-0.743144825477398,-0.669130606358854,
1.04647355694969E-16));
#122252=DIRECTION('ref_axis',(0.669130606358854,-0.743144825477398,-1.33231393542051E-30));
#122253=DIRECTION('center_axis',(-0.743144825477406,-0.669130606358845,
0.));
#122254=DIRECTION('ref_axis',(0.669130606358845,-0.743144825477406,0.));
#122255=DIRECTION('center_axis',(-0.743144825477398,-0.669130606358854,
1.04647355694969E-16));
#122256=DIRECTION('ref_axis',(0.669130606358854,-0.743144825477398,-1.33231393542051E-30));
#122257=DIRECTION('center_axis',(0.643614221961228,0.579466481046758,-0.499979330205289));
#122258=DIRECTION('ref_axis',(0.372201885192673,0.33383492295096,0.866036951219373));
#122259=DIRECTION('center_axis',(-0.371576246276125,-0.334568754912021,
0.866022425483293));
#122260=DIRECTION('ref_axis',(0.918982131463643,-6.34168247799913E-15,0.394299178353873));
#122261=DIRECTION('center_axis',(-0.371576252946094,-0.334568760917662,
0.866022420301323));
#122262=DIRECTION('ref_axis',(-0.669130606357769,0.743144825478375,8.3922370166019E-13));
#122263=DIRECTION('center_axis',(0.404512553894235,0.293895573516223,0.866022508719914));
#122264=DIRECTION('ref_axis',(0.587785252291253,-0.809016994375834,8.74191359985202E-13));
#122265=DIRECTION('center_axis',(0.700605801485921,0.509057044367645,0.500012436349285));
#122266=DIRECTION('ref_axis',(-0.405100113149077,-0.293099122184537,0.86601778440241));
#122267=DIRECTION('center_axis',(-0.404512560891477,-0.293895578600006,
-0.86602250372631));
#122268=DIRECTION('ref_axis',(-0.906035256115479,9.01705582438248E-15,0.423202214875771));
#122269=DIRECTION('center_axis',(-0.80901699437495,-0.58778525229247,0.));
#122270=DIRECTION('ref_axis',(0.58778525229247,-0.80901699437495,0.));
#122271=DIRECTION('center_axis',(0.809016994374951,0.587785252292469,-1.13923270769253E-16));
#122272=DIRECTION('ref_axis',(-0.587785252292469,0.80901699437495,3.40207274335237E-32));
#122273=DIRECTION('center_axis',(0.80901699437495,0.58778525229247,0.));
#122274=DIRECTION('ref_axis',(-0.58778525229247,0.80901699437495,0.));
#122275=DIRECTION('center_axis',(0.809016994374951,0.587785252292469,-1.13923270769253E-16));
#122276=DIRECTION('ref_axis',(-0.587785252292469,0.80901699437495,3.40207274335237E-32));
#122277=DIRECTION('center_axis',(-0.809016994374976,-0.587785252292434,
0.));
#122278=DIRECTION('ref_axis',(0.587785252292434,-0.809016994374976,0.));
#122279=DIRECTION('center_axis',(0.428717694262762,0.311481637390294,-0.848045003637592));
#122280=DIRECTION('ref_axis',(-0.89244205802627,-6.91749752624164E-15,-0.451162025292284));
#122281=DIRECTION('center_axis',(-0.404512670528675,-0.293895658256101,
0.866022425483297));
#122282=DIRECTION('ref_axis',(0.906035197473499,-2.43383441813702E-15,0.423202340422591));
#122283=DIRECTION('center_axis',(-0.428717684114261,-0.311481603277307,
0.848045021297515));
#122284=DIRECTION('ref_axis',(-0.688609525582324,-0.494977266823274,-0.529919264233192));
#122285=DIRECTION('center_axis',(0.428717648856936,0.31148160440103,-0.848045038708641));
#122286=DIRECTION('ref_axis',(-0.892442084777727,-1.51672008863495E-15,
-0.451161972375314));
#122287=DIRECTION('center_axis',(-0.404512687916182,-0.293895657890621,
0.866022417485751));
#122288=DIRECTION('ref_axis',(-0.703293181145105,-0.505350078019966,-0.500000000000014));
#122289=DIRECTION('center_axis',(-0.700618669263857,-0.509071851162881,
0.4999793302053));
#122290=DIRECTION('ref_axis',(-0.403924952205241,-0.294660197700078,-0.866036951219372));
#122291=DIRECTION('center_axis',(-0.587589051772227,0.809159506053914,0.));
#122292=DIRECTION('ref_axis',(-0.809159506053914,-0.587589051772227,0.));
#122293=DIRECTION('center_axis',(0.809016994374951,0.587785252292469,-1.13923270769253E-16));
#122294=DIRECTION('ref_axis',(-0.587785252292469,0.80901699437495,3.40207274335237E-32));
#122295=DIRECTION('center_axis',(-0.80901699437495,-0.58778525229247,0.));
#122296=DIRECTION('ref_axis',(0.58778525229247,-0.80901699437495,0.));
#122297=DIRECTION('center_axis',(-2.54740177659163E-16,-8.27701011433311E-17,
-1.));
#122298=DIRECTION('ref_axis',(-1.,2.9359879547111E-33,2.25664243350207E-16));
#122299=DIRECTION('center_axis',(-0.587981418248456,0.808874435122371,0.));
#122300=DIRECTION('ref_axis',(-0.808874435122371,-0.587981418248456,0.));
#122301=DIRECTION('center_axis',(-0.428718069290576,-0.31148190986395,-0.848044713969298));
#122302=DIRECTION('ref_axis',(-0.892441837073373,-7.49535211974272E-15,
0.451162462358188));
#122303=DIRECTION('center_axis',(-0.428717648856939,-0.311481604401032,
0.848045038708639));
#122304=DIRECTION('ref_axis',(0.892442084777726,6.53865308856261E-16,0.451161972375317));
#122305=DIRECTION('center_axis',(-0.428718080852829,-0.3114819494368,-0.848044693589269));
#122306=DIRECTION('ref_axis',(0.688740099746409,0.4947955622233,-0.52991926423318));
#122307=DIRECTION('center_axis',(-0.428718122142682,-0.311481948263282,
-0.848044673146741));
#122308=DIRECTION('ref_axis',(-0.892441805934785,-7.52869580075203E-16,
0.451162523953242));
#122309=DIRECTION('center_axis',(0.428717684276781,0.311481603322996,-0.848045021198575));
#122310=DIRECTION('ref_axis',(-0.683543400925772,-0.501950189207415,-0.529919264233213));
#122311=DIRECTION('center_axis',(-0.428717694262774,-0.311481637390302,
0.848045003637583));
#122312=DIRECTION('ref_axis',(0.892442058026264,2.33582750500883E-15,0.451162025292297));
#122313=DIRECTION('center_axis',(-0.587576360591347,0.809168721883284,4.42105189882562E-14));
#122314=DIRECTION('ref_axis',(-0.809168721883284,-0.587576360591347,9.93302310845174E-28));
#122315=DIRECTION('center_axis',(-0.80901699437495,-0.58778525229247,4.42022290584717E-14));
#122316=DIRECTION('ref_axis',(0.58778525229247,-0.80901699437495,3.78613142600248E-30));
#122317=DIRECTION('center_axis',(-2.54740177659163E-16,-8.27701011433311E-17,
-1.));
#122318=DIRECTION('ref_axis',(-1.,1.66692058590397E-33,2.40228573745067E-16));
#122319=DIRECTION('center_axis',(-0.587994104813612,0.80886521293998,-1.20677258718682E-14));
#122320=DIRECTION('ref_axis',(-0.80886521293998,-0.587994104813612,1.51939136976245E-28));
#122321=DIRECTION('center_axis',(-0.809016994374951,-0.587785252292469,
1.13923270769253E-16));
#122322=DIRECTION('ref_axis',(0.587785252292469,-0.809016994374951,1.93507240347744E-30));
#122323=DIRECTION('center_axis',(-0.700641118228684,-0.509008435041272,
-0.500012436349432));
#122324=DIRECTION('ref_axis',(0.40393664947362,0.294700492552831,-0.866017784402344));
#122325=DIRECTION('center_axis',(0.428718122142701,0.311481948263287,0.848044673146729));
#122326=DIRECTION('ref_axis',(0.892441805934776,-6.12251068898412E-15,-0.45116252395326));
#122327=DIRECTION('center_axis',(0.40451254409338,0.293895578897687,0.866022511471553));
#122328=DIRECTION('ref_axis',(0.69798874133117,0.51265165265994,-0.499999999999961));
#122329=DIRECTION('center_axis',(-0.404512560891434,-0.293895578599982,
-0.866022503726338));
#122330=DIRECTION('ref_axis',(-0.9060352561155,-6.08383211411716E-15,0.423202214875727));
#122331=DIRECTION('center_axis',(0.428718080657259,0.311481949375618,0.848044693710609));
#122332=DIRECTION('ref_axis',(0.683410939236706,0.502130522400415,-0.529919264233232));
#122333=DIRECTION('center_axis',(0.42871806929053,0.311481909863937,0.848044713969325));
#122334=DIRECTION('ref_axis',(0.892441837073399,2.26869662838081E-15,-0.451162462358136));
#122335=DIRECTION('center_axis',(-0.80901699437495,-0.58778525229247,0.));
#122336=DIRECTION('ref_axis',(0.58778525229247,-0.80901699437495,0.));
#122337=DIRECTION('center_axis',(0.809016994374976,0.587785252292434,0.));
#122338=DIRECTION('ref_axis',(-0.587785252292434,0.809016994374976,0.));
#122339=DIRECTION('center_axis',(-0.809016994374951,-0.587785252292469,
1.13923270769253E-16));
#122340=DIRECTION('ref_axis',(0.587785252292469,-0.809016994374951,1.93507240347744E-30));
#122341=DIRECTION('center_axis',(-0.80901699437495,-0.58778525229247,-3.2114799243612E-14));
#122342=DIRECTION('ref_axis',(0.58778525229247,-0.80901699437495,-4.13565546558353E-30));
#122343=DIRECTION('center_axis',(-0.809016994374951,-0.587785252292469,
1.13923270769253E-16));
#122344=DIRECTION('ref_axis',(0.587785252292469,-0.809016994374951,1.93507240347744E-30));
#122345=DIRECTION('center_axis',(0.700659176689548,0.509016097474346,-0.499979330205472));
#122346=DIRECTION('ref_axis',(0.405058175792506,0.293100449243017,0.866036951219282));
#122347=DIRECTION('center_axis',(-0.404512670528692,-0.293895658256113,
0.866022425483285));
#122348=DIRECTION('ref_axis',(0.906035197473489,5.57797719073592E-15,0.423202340422612));
#122349=DIRECTION('center_axis',(-0.404512677787103,-0.29389566352967,0.866022420303287));
#122350=DIRECTION('ref_axis',(-0.587785252285307,0.809016994380154,5.10527751848768E-12));
#122351=DIRECTION('center_axis',(0.433017044457923,0.250002507181456,0.866022508721287));
#122352=DIRECTION('ref_axis',(0.500000000003501,-0.866025403782417,-2.34283284476153E-12));
#122353=DIRECTION('center_axis',(0.749978760162693,0.43303512882966,0.500012436349646));
#122354=DIRECTION('ref_axis',(-0.433518133171605,-0.249149002226608,0.866017784402198));
#122355=DIRECTION('center_axis',(-0.433017051950273,-0.250002511507195,
-0.866022503726312));
#122356=DIRECTION('ref_axis',(-0.894424794863786,-9.37039710670596E-16,
0.447218387740122));
#122357=DIRECTION('center_axis',(-0.86602540378444,-0.499999999999998,-6.09762352041363E-14));
#122358=DIRECTION('ref_axis',(0.499999999999998,-0.86602540378444,-8.28350179725319E-28));
#122359=DIRECTION('center_axis',(0.866025403784442,0.499999999999995,-1.21951018649011E-16));
#122360=DIRECTION('ref_axis',(-0.499999999999995,0.866025403784441,2.67488359253536E-33));
#122361=DIRECTION('center_axis',(0.866025403784433,0.50000000000001,1.36592399683214E-14));
#122362=DIRECTION('ref_axis',(-0.50000000000001,0.866025403784433,-1.33215113601878E-31));
#122363=DIRECTION('center_axis',(0.866025403784442,0.499999999999995,-1.21951018649011E-16));
#122364=DIRECTION('ref_axis',(-0.499999999999995,0.866025403784441,2.67488359253536E-33));
#122365=DIRECTION('center_axis',(-0.86602540378444,-0.499999999999998,0.));
#122366=DIRECTION('ref_axis',(0.499999999999998,-0.86602540378444,0.));
#122367=DIRECTION('center_axis',(0.45892783076861,0.264962106632875,-0.848045003637594));
#122368=DIRECTION('ref_axis',(-0.879478602053341,-1.44813680787485E-15,
-0.475938429348064));
#122369=DIRECTION('center_axis',(-0.43301716931323,-0.250002579266683,0.866022425483292));
#122370=DIRECTION('ref_axis',(0.894424730216411,5.21485729842101E-15,0.447218517033117));
#122371=DIRECTION('center_axis',(-0.458927817107387,-0.264962073772023,
0.8480450212975));
#122372=DIRECTION('ref_axis',(-0.736576463613238,-0.420286434048956,-0.529919264233174));
#122373=DIRECTION('center_axis',(0.45892778216319,0.264962078570523,-0.848045038708655));
#122374=DIRECTION('ref_axis',(-0.879478631391258,-5.23853710775596E-15,
-0.475938375135017));
#122375=DIRECTION('center_axis',(-0.433017186566647,-0.250002577086723,
0.866022417485773));
#122376=DIRECTION('ref_axis',(-0.752263934577883,-0.429067561968314,-0.49999999999997));
#122377=DIRECTION('center_axis',(-0.74999310518157,-0.433048509462502,0.499979330205172));
#122378=DIRECTION('ref_axis',(-0.43251258670403,-0.25082436377896,-0.866036951219444));
#122379=DIRECTION('center_axis',(-0.499789977759954,0.866146626230631,0.));
#122380=DIRECTION('ref_axis',(-0.866146626230631,-0.499789977759954,0.));
#122381=DIRECTION('center_axis',(0.866025403784442,0.499999999999995,-1.21951018649011E-16));
#122382=DIRECTION('ref_axis',(-0.499999999999995,0.866025403784441,2.67488359253536E-33));
#122383=DIRECTION('center_axis',(-0.866025403784457,-0.499999999999969,
0.));
#122384=DIRECTION('ref_axis',(0.499999999999969,-0.866025403784457,0.));
#122385=DIRECTION('center_axis',(-2.62767925538921E-16,-7.04084534449545E-17,
-1.));
#122386=DIRECTION('ref_axis',(-1.,2.9359879547111E-33,2.25664243350207E-16));
#122387=DIRECTION('center_axis',(-0.500209992837911,0.865904130412309,0.));
#122388=DIRECTION('ref_axis',(-0.865904130412309,-0.500209992837911,0.));
#122389=DIRECTION('center_axis',(-0.458928232223204,-0.264962338412793,
-0.848044713969322));
#122390=DIRECTION('ref_axis',(-0.879478359737744,-1.81174991810093E-15,
0.475938877118698));
#122391=DIRECTION('center_axis',(-0.45892778216322,-0.264962078570532,0.848045038708636));
#122392=DIRECTION('ref_axis',(0.879478631391242,-3.91934596708905E-15,0.475938375135046));
#122393=DIRECTION('center_axis',(-0.458928247862902,-0.264962376552842,
-0.848044693589292));
#122394=DIRECTION('ref_axis',(0.73668732915428,0.420092076166699,-0.529919264233228));
#122395=DIRECTION('center_axis',(-0.458928288799617,-0.264962371077283,
-0.848044673146739));
#122396=DIRECTION('ref_axis',(-0.879478325588526,-1.55521142283728E-15,
0.475938940222381));
#122397=DIRECTION('center_axis',(0.458927817276937,0.264962073795002,-0.848045021198567));
#122398=DIRECTION('ref_axis',(-0.732266960571272,-0.427750712273227,-0.529919264233202));
#122399=DIRECTION('center_axis',(-0.458927830768617,-0.264962106632871,
0.848045003637592));
#122400=DIRECTION('ref_axis',(0.879478602053337,-4.79936374009227E-16,0.47593842934807));
#122401=DIRECTION('center_axis',(-0.499776392786171,0.866154464985111,0.));
#122402=DIRECTION('ref_axis',(-0.86615446498511,-0.499776392786171,0.));
#122403=DIRECTION('center_axis',(-0.866025403784433,-0.50000000000001,-1.36592399683221E-14));
#122404=DIRECTION('ref_axis',(0.50000000000001,-0.866025403784433,1.85779939211817E-28));
#122405=DIRECTION('center_axis',(-2.62767925538921E-16,-7.04084534449545E-17,
-1.));
#122406=DIRECTION('ref_axis',(-1.,1.97946819576097E-33,2.40228573745067E-16));
#122407=DIRECTION('center_axis',(-0.500223573885299,0.865896284857153,3.67572504895883E-15));
#122408=DIRECTION('ref_axis',(-0.865896284857153,-0.500223573885299,4.46977350782273E-29));
#122409=DIRECTION('center_axis',(-0.866025403784442,-0.499999999999995,
1.21951018649011E-16));
#122410=DIRECTION('ref_axis',(0.499999999999995,-0.866025403784442,2.10506284754485E-30));
#122411=DIRECTION('center_axis',(-0.750008802379564,-0.432983094185751,
-0.500012436347842));
#122412=DIRECTION('ref_axis',(0.432528431882832,0.250863215139549,-0.866017784403315));
#122413=DIRECTION('center_axis',(0.458928288799688,0.264962371077179,0.848044673146733));
#122414=DIRECTION('ref_axis',(0.879478325588494,-3.39387948166673E-15,-0.475938940222439));
#122415=DIRECTION('center_axis',(0.433017035278663,0.250002513553368,0.866022511471541));
#122416=DIRECTION('ref_axis',(0.747751775424751,0.436883602746915,-0.500000000000008));
#122417=DIRECTION('center_axis',(-0.43301705195022,-0.250002511507164,-0.866022503726347));
#122418=DIRECTION('ref_axis',(-0.894424794863815,-4.94594594567521E-15,
0.447218387740065));
#122419=DIRECTION('center_axis',(0.458928247651838,0.264962376530043,0.848044693710635));
#122420=DIRECTION('ref_axis',(0.732154074451793,0.427943903634897,-0.529919264233113));
#122421=DIRECTION('center_axis',(0.458928232223194,0.264962338412787,0.848044713969329));
#122422=DIRECTION('ref_axis',(0.87947835973775,5.0288465242107E-15,-0.475938877118687));
#122423=DIRECTION('center_axis',(-0.866025403784433,-0.50000000000001,0.));
#122424=DIRECTION('ref_axis',(0.50000000000001,-0.866025403784433,0.));
#122425=DIRECTION('center_axis',(0.866025403784433,0.50000000000001,0.));
#122426=DIRECTION('ref_axis',(-0.50000000000001,0.866025403784433,0.));
#122427=DIRECTION('center_axis',(-0.866025403784442,-0.499999999999995,
1.21951018649011E-16));
#122428=DIRECTION('ref_axis',(0.499999999999995,-0.866025403784442,2.10506284754485E-30));
#122429=DIRECTION('center_axis',(-0.866025403784433,-0.50000000000001,0.));
#122430=DIRECTION('ref_axis',(0.50000000000001,-0.866025403784433,0.));
#122431=DIRECTION('center_axis',(-0.866025403784442,-0.499999999999995,
1.21951018649011E-16));
#122432=DIRECTION('ref_axis',(0.499999999999995,-0.866025403784442,2.10506284754485E-30));
#122433=DIRECTION('center_axis',(0.750027562855788,0.432988827019605,-0.499979330205554));
#122434=DIRECTION('ref_axis',(0.433476564278272,0.24915470564377,0.866036951219214));
#122435=DIRECTION('center_axis',(-0.433017169313196,-0.25000257926671,0.866022425483301));
#122436=DIRECTION('ref_axis',(0.894424730216427,1.90878151355965E-15,0.447218517033085));
#122437=DIRECTION('center_axis',(-0.433017177086037,-0.250002583754367,
0.866022420301334));
#122438=DIRECTION('ref_axis',(-0.500000000002471,0.866025403783012,-1.64347974908538E-12));
#122439=DIRECTION('center_axis',(0.456777309663355,0.203370361060154,0.866022508725362));
#122440=DIRECTION('ref_axis',(0.406736643069877,-0.913545457645238,3.70657136640272E-12));
#122441=DIRECTION('center_axis',(0.791134794599999,0.352268789802096,0.500012436349921));
#122442=DIRECTION('ref_axis',(0.457186437788949,0.202469153702906,-0.866017784402076));
#122443=DIRECTION('center_axis',(-0.456777317573304,-0.203370364581847,
-0.866022503726308));
#122444=DIRECTION('ref_axis',(-0.884507036382085,-1.36888255260538E-16,
0.466526850878469));
#122445=DIRECTION('center_axis',(-0.913545457642594,-0.406736643075817,
0.));
#122446=DIRECTION('ref_axis',(0.406736643075817,-0.913545457642593,0.));
#122447=DIRECTION('center_axis',(0.913545457642603,0.406736643075795,-1.28642645648559E-16));
#122448=DIRECTION('ref_axis',(-0.406736643075795,0.913545457642603,1.45091416765994E-32));
#122449=DIRECTION('center_axis',(0.913545457642598,0.406736643075807,0.));
#122450=DIRECTION('ref_axis',(-0.406736643075807,0.913545457642598,0.));
#122451=DIRECTION('center_axis',(0.913545457642603,0.406736643075795,-1.28642645648559E-16));
#122452=DIRECTION('ref_axis',(-0.406736643075795,0.913545457642603,1.45091416765994E-32));
#122453=DIRECTION('center_axis',(-0.913545457642603,-0.406736643075797,
0.));
#122454=DIRECTION('ref_axis',(0.406736643075797,-0.913545457642603,0.));
#122455=DIRECTION('center_axis',(0.484109857923767,0.215539595588305,-0.848045003637578));
#122456=DIRECTION('ref_axis',(-0.868458021515997,-1.32153558682304E-15,
-0.49576271024001));
#122457=DIRECTION('center_axis',(-0.456777441376074,-0.20337041970247,0.866022425483295));
#122458=DIRECTION('ref_axis',(0.884506966812058,2.53897267290044E-15,0.466526982779059));
#122459=DIRECTION('center_axis',(-0.484109840902121,-0.215539564336208,
0.848045021297502));
#122460=DIRECTION('ref_axis',(-0.776473315744763,-0.340990855201216,-0.52991926423322));
#122461=DIRECTION('center_axis',(0.484109806651284,0.215539572760325,-0.848045038708649));
#122462=DIRECTION('ref_axis',(-0.86845805294996,4.78172523366081E-17,-0.4957626551752));
#122463=DIRECTION('center_axis',(-0.456777458307931,-0.203370415729123,
0.866022417485777));
#122464=DIRECTION('ref_axis',(-0.792992726927602,-0.348084091908765,-0.499999999999977));
#122465=DIRECTION('center_axis',(-0.791150459692809,-0.352280597671166,
0.499979330205063));
#122466=DIRECTION('ref_axis',(0.456361522800706,0.204240445625793,0.866036951219518));
#122467=DIRECTION('center_axis',(-0.406515100163568,0.913644062717536,0.));
#122468=DIRECTION('ref_axis',(-0.913644062717536,-0.406515100163568,0.));
#122469=DIRECTION('center_axis',(0.913545457642603,0.406736643075795,-1.28642645648559E-16));
#122470=DIRECTION('ref_axis',(-0.406736643075795,0.913545457642603,1.45091416765994E-32));
#122471=DIRECTION('center_axis',(-0.913545457642603,-0.406736643075797,
0.));
#122472=DIRECTION('ref_axis',(0.406736643075797,-0.913545457642603,0.));
#122473=DIRECTION('center_axis',(-2.6945955253847E-16,-5.7275395996719E-17,
-1.));
#122474=DIRECTION('ref_axis',(-1.,2.74025542439703E-33,2.25664243350207E-16));
#122475=DIRECTION('center_axis',(-0.406958162070199,0.913446798847336,0.));
#122476=DIRECTION('ref_axis',(-0.913446798847336,-0.406958162070199,0.));
#122477=DIRECTION('center_axis',(-0.484110281406756,-0.215539784135086,
-0.8480447139693));
#122478=DIRECTION('ref_axis',(-0.868457761888263,-2.07453665764236E-15,
0.495763165045598));
#122479=DIRECTION('center_axis',(-0.484109806651301,-0.215539572760332,
0.848045038708637));
#122480=DIRECTION('ref_axis',(0.86845805294995,-4.51368237441253E-15,0.495762655175218));
#122481=DIRECTION('center_axis',(-0.484110300944432,-0.215539820438308,
-0.848044693589267));
#122482=DIRECTION('ref_axis',(0.776563258047416,0.340785973369427,-0.52991926423318));
#122483=DIRECTION('center_axis',(-0.484110341087582,-0.215539810706759,
-0.848044673146739));
#122484=DIRECTION('ref_axis',(-0.868457725299282,6.1582383090763E-16,0.495763229140682));
#122485=DIRECTION('center_axis',(0.484109841073423,0.215539564340702,-0.848045021198572));
#122486=DIRECTION('ref_axis',(-0.772967650153761,-0.348864709035361,-0.52991926423319));
#122487=DIRECTION('center_axis',(-0.484109857923745,-0.215539595588295,
0.848045003637594));
#122488=DIRECTION('ref_axis',(0.868458021516011,-2.89436985092629E-15,0.495762710239986));
#122489=DIRECTION('center_axis',(-0.406500770236713,0.913650438514074,0.));
#122490=DIRECTION('ref_axis',(-0.913650438514073,-0.406500770236713,0.));
#122491=DIRECTION('center_axis',(-0.913545457642598,-0.406736643075807,
0.));
#122492=DIRECTION('ref_axis',(0.406736643075807,-0.913545457642598,0.));
#122493=DIRECTION('center_axis',(-2.6945955253847E-16,-5.7275395996719E-17,
-1.));
#122494=DIRECTION('ref_axis',(-1.,1.97946819576097E-33,2.40228573745067E-16));
#122495=DIRECTION('center_axis',(-0.406972488803014,0.913440415876964,0.));
#122496=DIRECTION('ref_axis',(-0.913440415876964,-0.406972488803014,0.));
#122497=DIRECTION('center_axis',(-0.913545457642603,-0.406736643075795,
1.28642645648559E-16));
#122498=DIRECTION('ref_axis',(0.406736643075795,-0.913545457642603,1.67756362845828E-30));
#122499=DIRECTION('center_axis',(-0.791159233141683,-0.352213899942492,
-0.500012436347302));
#122500=DIRECTION('ref_axis',(0.456381342239291,0.204277427907535,-0.866017784403614));
#122501=DIRECTION('center_axis',(0.484110341087604,0.215539810706711,0.848044673146739));
#122502=DIRECTION('ref_axis',(0.868457725299272,5.31136787545075E-15,-0.4957632291407));
#122503=DIRECTION('center_axis',(0.456777301208103,0.203370368356831,0.866022511471525));
#122504=DIRECTION('ref_axis',(0.789322284583639,0.356328964665585,-0.500000000000017));
#122505=DIRECTION('center_axis',(-0.456777317573169,-0.203370364581866,
-0.866022503726375));
#122506=DIRECTION('ref_axis',(-0.884507036382156,-6.36152350155046E-15,
0.466526850878334));
#122507=DIRECTION('center_axis',(0.48411030073694,0.215539820426895,0.848044693710615));
#122508=DIRECTION('ref_axis',(0.77287557643918,0.349068641872047,-0.529919264233156));
#122509=DIRECTION('center_axis',(0.484110281406739,0.215539784135021,0.848044713969326));
#122510=DIRECTION('ref_axis',(0.868457761888278,-1.94242193778803E-15,-0.495763165045573));
#122511=DIRECTION('center_axis',(-0.913545457642598,-0.406736643075807,
0.));
#122512=DIRECTION('ref_axis',(0.406736643075807,-0.913545457642598,0.));
#122513=DIRECTION('center_axis',(0.913545457642598,0.406736643075807,0.));
#122514=DIRECTION('ref_axis',(-0.406736643075807,0.913545457642598,0.));
#122515=DIRECTION('center_axis',(-0.913545457642603,-0.406736643075795,
1.28642645648559E-16));
#122516=DIRECTION('ref_axis',(0.406736643075795,-0.913545457642603,1.67756362845828E-30));
#122517=DIRECTION('center_axis',(-0.913545457642598,-0.406736643075807,
1.11114268233636E-14));
#122518=DIRECTION('ref_axis',(0.406736643075807,-0.913545457642598,-1.92826049468501E-31));
#122519=DIRECTION('center_axis',(-0.913545457642603,-0.406736643075795,
1.28642645648559E-16));
#122520=DIRECTION('ref_axis',(0.406736643075795,-0.913545457642603,1.67756362845828E-30));
#122521=DIRECTION('center_axis',(0.791178490090852,0.352217640366497,-0.499979330204976));
#122522=DIRECTION('ref_axis',(0.457145692795309,0.202479170980695,0.866036951219558));
#122523=DIRECTION('center_axis',(-0.456777441376052,-0.203370419702461,
0.866022425483308));
#122524=DIRECTION('ref_axis',(0.884506966812071,-1.93472172084304E-15,0.466526982779036));
#122525=DIRECTION('center_axis',(-0.456777449576467,-0.203370423353516,
0.86602242030067));
#122526=DIRECTION('ref_axis',(-0.406736643078774,0.913545457641277,-1.88825332874541E-12));
#122527=DIRECTION('center_axis',(0.475533027092593,0.154510046711641,0.866022508719792));
#122528=DIRECTION('ref_axis',(0.309016994372452,-0.951056516295964,1.53857679358147E-12));
#122529=DIRECTION('center_axis',(0.823622990673448,0.267642920194726,0.500012436349103));
#122530=DIRECTION('ref_axis',(0.475845712132185,0.153571010753556,-0.866017784402575));
#122531=DIRECTION('center_axis',(-0.475533035318161,-0.154510049384248,
-0.866022503726303));
#122532=DIRECTION('ref_axis',(-0.876548788012425,-4.15617318960849E-15,
0.481313018974086));
#122533=DIRECTION('center_axis',(-0.951056516295146,-0.309016994374972,
0.));
#122534=DIRECTION('ref_axis',(0.309016994374972,-0.951056516295146,0.));
#122535=DIRECTION('center_axis',(0.951056516295156,0.309016994374942,-1.33924836902178E-16));
#122536=DIRECTION('ref_axis',(-0.309016994374942,0.951056516295155,-1.29861735441449E-32));
#122537=DIRECTION('center_axis',(0.951056516295148,0.309016994374964,-1.68837491218278E-14));
#122538=DIRECTION('ref_axis',(-0.309016994374964,0.951056516295148,-1.43380940262431E-28));
#122539=DIRECTION('center_axis',(0.951056516295156,0.309016994374942,-1.33924836902178E-16));
#122540=DIRECTION('ref_axis',(-0.309016994374942,0.951056516295155,5.50275392197254E-33));
#122541=DIRECTION('center_axis',(-0.951056516295146,-0.309016994374972,
0.));
#122542=DIRECTION('ref_axis',(0.309016994374972,-0.951056516295146,0.));
#122543=DIRECTION('center_axis',(0.503987876168977,0.163755587629901,-0.848045003637584));
#122544=DIRECTION('ref_axis',(-0.859649462041493,1.86435088897448E-15,-0.510884333691856));
#122545=DIRECTION('center_axis',(-0.475533164204401,-0.15451009126198,0.866022425483292));
#122546=DIRECTION('ref_axis',(0.876548714628841,-1.25657155782984E-15,0.481313152617426));
#122547=DIRECTION('center_axis',(-0.503987855974141,-0.163755558327407,
0.848045021297495));
#122548=DIRECTION('ref_axis',(-0.807862963766476,-0.257959309134166,-0.529919264233212));
#122549=DIRECTION('center_axis',(0.503987822791196,0.163755570286409,-0.848045038708654));
#122550=DIRECTION('ref_axis',(-0.859649495083708,-1.81880948564364E-15,
-0.510884278092727));
#122551=DIRECTION('center_axis',(-0.475533180627884,-0.154510085541378,
0.866022417485786));
#122552=DIRECTION('ref_axis',(-0.825033325010246,-0.263286939711361,-0.499999999999964));
#122553=DIRECTION('center_axis',(-0.823639804208727,-0.267653025932132,
0.499979330205143));
#122554=DIRECTION('ref_axis',(0.475210466540287,0.15541882644351,0.866036951219453));
#122555=DIRECTION('center_axis',(-0.308786358060986,0.951131423661017,0.));
#122556=DIRECTION('ref_axis',(-0.951131423661017,-0.308786358060986,0.));
#122557=DIRECTION('center_axis',(0.951056516295156,0.309016994374942,-1.33924836902178E-16));
#122558=DIRECTION('ref_axis',(-0.309016994374942,0.951056516295155,-1.29861735441449E-32));
#122559=DIRECTION('center_axis',(-0.951056516295162,-0.309016994374922,
0.));
#122560=DIRECTION('ref_axis',(0.309016994374922,-0.951056516295162,0.));
#122561=DIRECTION('center_axis',(-2.74741743792088E-16,-4.35148173242961E-17,
-1.));
#122562=DIRECTION('ref_axis',(-1.,2.34879036376888E-33,2.25664243350207E-16));
#122563=DIRECTION('center_axis',(-0.309247612517378,0.95098155300316,0.));
#122564=DIRECTION('ref_axis',(-0.95098155300316,-0.309247612517378,0.));
#122565=DIRECTION('center_axis',(-0.503988317040574,-0.163755730877723,
-0.848044713969324));
#122566=DIRECTION('ref_axis',(-0.859649189130472,-1.11108923047349E-15,
0.510884792910616));
#122567=DIRECTION('center_axis',(-0.503987822791213,-0.163755570286414,
0.848045038708643));
#122568=DIRECTION('ref_axis',(0.859649495083697,-1.4932809657743E-15,0.510884278092744));
#122569=DIRECTION('center_axis',(-0.503988340268045,-0.163755764933357,
-0.84804469358929));
#122570=DIRECTION('ref_axis',(0.80793099735763,0.257746148183087,-0.529919264233229));
#122571=DIRECTION('center_axis',(-0.503988379172003,-0.163755751065511,
-0.848044673146732));
#122572=DIRECTION('ref_axis',(-0.859649150669465,1.72876348210857E-15,0.510884857627693));
#122573=DIRECTION('center_axis',(0.503987856145422,0.163755558312599,-0.848045021198562));
#122574=DIRECTION('ref_axis',(-0.805199544416579,-0.266156471020048,-0.52991926423323));
#122575=DIRECTION('center_axis',(-0.503987876169011,-0.163755587629912,
0.848045003637562));
#122576=DIRECTION('ref_axis',(0.859649462041472,-9.84505827227631E-16,0.510884333691892));
#122577=DIRECTION('center_axis',(-0.308771440182777,0.951136266645034,0.));
#122578=DIRECTION('ref_axis',(-0.951136266645034,-0.308771440182777,0.));
#122579=DIRECTION('center_axis',(-0.951056516295148,-0.309016994374964,
5.19628367180465E-14));
#122580=DIRECTION('ref_axis',(0.309016994374964,-0.951056516295148,4.387849755876E-28));
#122581=DIRECTION('center_axis',(-2.74741743792088E-16,-4.35148173242961E-17,
-1.));
#122582=DIRECTION('ref_axis',(-1.,1.71901185421347E-33,2.40228573745067E-16));
#122583=DIRECTION('center_axis',(-0.309262527968948,0.950976702550728,-9.08207363789677E-15));
#122584=DIRECTION('ref_axis',(-0.950976702550728,-0.309262527968948,9.18332529948884E-29));
#122585=DIRECTION('center_axis',(-0.951056516295156,-0.309016994374942,
1.33924836902178E-16));
#122586=DIRECTION('ref_axis',(0.309016994374942,-0.951056516295156,3.08051195631577E-30));
#122587=DIRECTION('center_axis',(-0.823641557783683,-0.267585776505055,
-0.500012436349192));
#122588=DIRECTION('ref_axis',(0.475234043096222,0.15545353447593,-0.866017784402468));
#122589=DIRECTION('center_axis',(0.503988379172001,0.163755751065462,0.848044673146743));
#122590=DIRECTION('ref_axis',(0.859649150669468,-6.63213536595391E-16,-0.510884857627688));
#122591=DIRECTION('center_axis',(0.475533019435078,0.154510054855637,0.866022511471535));
#122592=DIRECTION('ref_axis',(0.822244813610695,0.271870311895752,-0.500000000000019));
#122593=DIRECTION('center_axis',(-0.475533035318099,-0.154510049384278,
-0.866022503726331));
#122594=DIRECTION('ref_axis',(-0.876548788012458,-3.21789385138784E-15,
0.481313018974027));
#122595=DIRECTION('center_axis',(0.503988340058086,0.163755764951276,0.848044693710607));
#122596=DIRECTION('ref_axis',(0.805129291880749,0.266368911005196,-0.529919264233251));
#122597=DIRECTION('center_axis',(0.503988317040564,0.16375573087773,0.848044713969329));
#122598=DIRECTION('ref_axis',(0.859649189130477,2.91164143962136E-15,-0.510884792910607));
#122599=DIRECTION('center_axis',(-0.951056516295148,-0.309016994374964,
5.19628367180465E-14));
#122600=DIRECTION('ref_axis',(0.309016994374964,-0.951056516295148,4.387849755876E-28));
#122601=DIRECTION('center_axis',(0.951056516295165,0.309016994374914,0.));
#122602=DIRECTION('ref_axis',(-0.309016994374914,0.951056516295164,0.));
#122603=DIRECTION('center_axis',(-0.951056516295156,-0.309016994374942,
1.33924836902178E-16));
#122604=DIRECTION('ref_axis',(0.309016994374942,-0.951056516295156,3.08051195631577E-30));
#122605=DIRECTION('center_axis',(-0.951056516295148,-0.309016994374964,
5.19628367180436E-14));
#122606=DIRECTION('ref_axis',(0.309016994374964,-0.951056516295148,4.43497354731716E-28));
#122607=DIRECTION('center_axis',(-0.951056516295156,-0.309016994374942,
1.33924836902178E-16));
#122608=DIRECTION('ref_axis',(0.309016994374942,-0.951056516295156,3.08051195631577E-30));
#122609=DIRECTION('center_axis',(0.823661100222813,0.267587483540049,-0.499979330205209));
#122610=DIRECTION('ref_axis',(0.475806237445136,0.153585232137957,0.866036951219423));
#122611=DIRECTION('center_axis',(-0.475533164204424,-0.154510091261983,
0.866022425483279));
#122612=DIRECTION('ref_axis',(0.876548714628828,1.92992104204874E-15,0.48131315261745));
#122613=DIRECTION('center_axis',(-0.475533172739555,-0.154510094035192,
0.866022420301858));
#122614=DIRECTION('ref_axis',(-0.30901699437591,0.951056516294841,-5.94450122003489E-13));
#122615=DIRECTION('center_axis',(0.489078705152277,0.103956887953192,0.866022508722296));
#122616=DIRECTION('ref_axis',(0.207911690817373,-0.978147600733888,2.09805926398475E-13));
#122617=DIRECTION('center_axis',(0.847087400905789,0.180084698747132,0.500012436349167));
#122618=DIRECTION('ref_axis',(0.489291521299429,0.102990311598153,-0.866017784402495));
#122619=DIRECTION('center_axis',(-0.48907871361637,-0.103956889752269,-0.866022503726313));
#122620=DIRECTION('ref_axis',(-0.870740345484703,-1.90004769966601E-15,
0.491743073916837));
#122621=DIRECTION('center_axis',(-0.978147600733807,-0.207911690817751,
0.));
#122622=DIRECTION('ref_axis',(0.207911690817752,-0.978147600733807,0.));
#122623=DIRECTION('center_axis',(0.978147600733807,0.207911690817753,-1.37739719617122E-16));
#122624=DIRECTION('ref_axis',(-0.207911690817753,0.978147600733807,6.2795738784361E-33));
#122625=DIRECTION('center_axis',(0.978147600733806,0.207911690817757,2.83991567709912E-15));
#122626=DIRECTION('ref_axis',(-0.207911690817757,0.978147600733806,-3.75217731718872E-32));
#122627=DIRECTION('center_axis',(0.978147600733807,0.207911690817753,-1.37739719617122E-16));
#122628=DIRECTION('ref_axis',(-0.207911690817753,0.978147600733807,1.15415498391972E-33));
#122629=DIRECTION('center_axis',(-0.978147600733807,-0.207911690817751,
0.));
#122630=DIRECTION('ref_axis',(0.207911690817752,-0.978147600733807,0.));
#122631=DIRECTION('center_axis',(0.518344097776653,0.110177439185354,-0.848045003637581));
#122632=DIRECTION('ref_axis',(-0.853239582811869,3.05350236707336E-15,-0.521519140898039));
#122633=DIRECTION('center_axis',(-0.489078846173993,-0.103956917928312,
0.866022425483291));
#122634=DIRECTION('ref_axis',(0.87074026939378,2.35244089688217E-16,0.491743208652694));
#122635=DIRECTION('center_axis',(-0.518344074628207,-0.110177412160433,
0.848045021297489));
#122636=DIRECTION('ref_axis',(-0.830401496086228,-0.172101506943537,-0.529919264233258));
#122637=DIRECTION('center_axis',(0.518344042878396,0.110177427516369,-0.848045038708649));
#122638=DIRECTION('ref_axis',(-0.853239616987304,-1.56305751275697E-15,
-0.521519084984776));
#122639=DIRECTION('center_axis',(-0.489078861910133,-0.103956910519561,
0.866022417485781));
#122640=DIRECTION('ref_axis',(-0.848034685338687,-0.175605160694559,-0.499999999999952));
#122641=DIRECTION('center_axis',(-0.847105178671993,-0.180092991630926,
0.499979330205273));
#122642=DIRECTION('ref_axis',(0.488852904973924,0.104894406052942,0.866036951219379));
#122643=DIRECTION('center_axis',(-0.207674488001825,0.978197989689807,-1.33614410777024E-14));
#122644=DIRECTION('ref_axis',(-0.978197989689807,-0.207674488001825,-1.57019667026149E-28));
#122645=DIRECTION('center_axis',(0.978147600733807,0.207911690817753,-1.37739719617122E-16));
#122646=DIRECTION('ref_axis',(-0.207911690817753,0.978147600733807,6.2795738784361E-33));
#122647=DIRECTION('center_axis',(-0.978147600733807,-0.207911690817751,
0.));
#122648=DIRECTION('ref_axis',(0.207911690817751,-0.978147600733807,0.));
#122649=DIRECTION('center_axis',(-2.78556626507032E-16,-2.92774812072074E-17,
-1.));
#122650=DIRECTION('ref_axis',(-1.,-1.56586024251259E-33,2.25664243350207E-16));
#122651=DIRECTION('center_axis',(-0.208148881407613,0.978097154258594,0.));
#122652=DIRECTION('ref_axis',(-0.978097154258594,-0.208148881407613,0.));
#122653=DIRECTION('center_axis',(-0.518344551206596,-0.110177535564893,
-0.848044713969304));
#122654=DIRECTION('ref_axis',(-0.853239300541031,-1.51561929168402E-15,
0.521519602711396));
#122655=DIRECTION('center_axis',(-0.518344042878388,-0.110177427516367,
0.848045038708654));
#122656=DIRECTION('ref_axis',(0.85323961698731,-2.50985335815255E-15,0.521519084984768));
#122657=DIRECTION('center_axis',(-0.518344577867011,-0.110177567003933,
-0.848044693589297));
#122658=DIRECTION('ref_axis',(0.830446875604274,0.171882402222111,-0.5299192642332));
#122659=DIRECTION('center_axis',(-0.51834461510783,-0.110177549147536,-0.848044673146738));
#122660=DIRECTION('ref_axis',(-0.853239260760977,2.64094694942535E-15,0.521519667794094));
#122661=DIRECTION('center_axis',(0.518344074797617,0.110177412124785,-0.848045021198573));
#122662=DIRECTION('ref_axis',(-0.828609503967038,-0.180532167023046,-0.529919264233206));
#122663=DIRECTION('center_axis',(-0.518344097776682,-0.11017743918536,0.848045003637563));
#122664=DIRECTION('ref_axis',(0.85323958281185,1.36926545915298E-15,0.521519140898069));
#122665=DIRECTION('center_axis',(-0.207659145615642,0.978201246800566,-2.01562116103747E-15));
#122666=DIRECTION('ref_axis',(-0.978201246800566,-0.207659145615642,1.35421654966406E-29));
#122667=DIRECTION('center_axis',(-0.978147600733806,-0.207911690817757,
-2.83991567709928E-15));
#122668=DIRECTION('ref_axis',(0.207911690817757,-0.978147600733806,-6.5334247463116E-32));
#122669=DIRECTION('center_axis',(-2.78556626507032E-16,-2.92774812072074E-17,
-1.));
#122670=DIRECTION('ref_axis',(-1.,1.27623607358273E-33,2.40228573745067E-16));
#122671=DIRECTION('center_axis',(-0.208164222161104,0.978093889466682,0.));
#122672=DIRECTION('ref_axis',(-0.978093889466682,-0.208164222161104,0.));
#122673=DIRECTION('center_axis',(-0.978147600733807,-0.207911690817753,
1.37739719617122E-16));
#122674=DIRECTION('ref_axis',(0.207911690817753,-0.978147600733807,5.37037489645435E-31));
#122675=DIRECTION('center_axis',(-0.847099893161371,-0.180025927303929,
-0.500012436349692));
#122676=DIRECTION('ref_axis',(0.488879980359381,0.104926459498552,-0.866017784402208));
#122677=DIRECTION('center_axis',(0.518344615107833,0.110177549147492,0.848044673146742));
#122678=DIRECTION('ref_axis',(0.853239260760976,-2.77194105736839E-15,-0.521519667794094));
#122679=DIRECTION('center_axis',(0.489078698392183,0.103956896853947,0.866022511471559));
#122680=DIRECTION('ref_axis',(0.846158656399947,0.184432991082058,-0.499999999999962));
#122681=DIRECTION('center_axis',(-0.489078713616272,-0.103956889752271,
-0.866022503726368));
#122682=DIRECTION('ref_axis',(-0.870740345484759,-1.01855317828021E-15,
0.491743073916738));
#122683=DIRECTION('center_axis',(0.518344577661094,0.110177567039033,0.848044693710597));
#122684=DIRECTION('ref_axis',(0.828561842309643,0.180750786617714,-0.529919264233268));
#122685=DIRECTION('center_axis',(0.518344551206575,0.110177535564859,0.848044713969322));
#122686=DIRECTION('ref_axis',(0.853239300541045,-5.67982937678162E-16,-0.521519602711372));
#122687=DIRECTION('center_axis',(-0.978147600733806,-0.207911690817757,
0.));
#122688=DIRECTION('ref_axis',(0.207911690817757,-0.978147600733806,0.));
#122689=DIRECTION('center_axis',(0.978147600733806,0.20791169081776,0.));
#122690=DIRECTION('ref_axis',(-0.20791169081776,0.978147600733805,0.));
#122691=DIRECTION('center_axis',(-0.978147600733807,-0.207911690817753,
1.37739719617122E-16));
#122692=DIRECTION('ref_axis',(0.207911690817753,-0.978147600733807,5.37037489645435E-31));
#122693=DIRECTION('center_axis',(-0.978147600733806,-0.207911690817757,
0.));
#122694=DIRECTION('ref_axis',(0.207911690817757,-0.978147600733806,0.));
#122695=DIRECTION('center_axis',(-0.978147600733807,-0.207911690817753,
1.37739719617122E-16));
#122696=DIRECTION('ref_axis',(0.207911690817753,-0.978147600733807,5.37037489645435E-31));
#122697=DIRECTION('center_axis',(0.847119506978269,0.180025582247972,-0.499979330205933));
#122698=DIRECTION('ref_axis',(0.489253749394679,0.103008581324964,0.866036951218981));
#122699=DIRECTION('center_axis',(-0.489078846173999,-0.103956917928286,
0.866022425483291));
#122700=DIRECTION('ref_axis',(0.870740269393778,-3.33045470606309E-16,0.491743208652698));
#122701=DIRECTION('center_axis',(-0.489078854957332,-0.103956919795235,
0.866022420298869));
#122702=DIRECTION('ref_axis',(-0.207911690817491,0.978147600733863,1.39870616944244E-13));
#122703=DIRECTION('center_axis',(0.497265934579216,0.0522647557776183,0.866022508720509));
#122704=DIRECTION('ref_axis',(0.10452846327069,-0.994521895367954,-1.74838271998628E-12));
#122705=DIRECTION('center_axis',(0.861270944309505,0.0905534316547599,0.500012436349098));
#122706=DIRECTION('ref_axis',(0.497376550150645,0.0512812291070752,-0.866017784402555));
#122707=DIRECTION('center_axis',(-0.497265943181917,-0.0522647566818157,
-0.866022503726311));
#122708=DIRECTION('ref_axis',(-0.867207748104378,1.34059683546342E-16,0.497946504785137));
#122709=DIRECTION('center_axis',(-0.994521895368276,-0.104528463267628,
0.));
#122710=DIRECTION('ref_axis',(0.104528463267628,-0.994521895368276,0.));
#122711=DIRECTION('center_axis',(0.994521895368274,0.104528463267647,-1.40045497140052E-16));
#122712=DIRECTION('ref_axis',(-0.104528463267647,0.994521895368274,4.46085091676035E-33));
#122713=DIRECTION('center_axis',(0.994521895368276,0.104528463267629,1.42777936329246E-15));
#122714=DIRECTION('ref_axis',(-0.104528463267629,0.994521895368276,-1.01175703524978E-30));
#122715=DIRECTION('center_axis',(0.994521895368274,0.104528463267647,-1.40045497140052E-16));
#122716=DIRECTION('ref_axis',(-0.104528463267647,0.994521895368274,4.46085091676035E-33));
#122717=DIRECTION('center_axis',(-0.994521895368276,-0.104528463267627,
0.));
#122718=DIRECTION('ref_axis',(0.104528463267627,-0.994521895368276,0.));
#122719=DIRECTION('center_axis',(0.527021232978628,0.0553921636609795,-0.848045003637568));
#122720=DIRECTION('ref_axis',(-0.849349030019368,-9.93784749494393E-16,
-0.527831625809934));
#122721=DIRECTION('center_axis',(-0.497266077958573,-0.0522647708473854,
0.866022425483295));
#122722=DIRECTION('ref_axis',(0.867207670398082,4.13270435684635E-16,0.497946640115918));
#122723=DIRECTION('center_axis',(-0.527021207132258,-0.0553921392020563,
0.8480450212975));
#122724=DIRECTION('ref_axis',(-0.843841975852909,-0.0843581245832878,-0.529919264233193));
#122725=DIRECTION('center_axis',(0.527021177161346,0.0553921577943468,-0.84804503870865));
#122726=DIRECTION('ref_axis',(-0.84934906486752,-5.14909852082013E-16,-0.527831569734768));
#122727=DIRECTION('center_axis',(-0.497266092833646,-0.0522647618386464,
0.866022417485777));
#122728=DIRECTION('ref_axis',(-0.861744800189479,-0.0859994148029189,-0.49999999999995));
#122729=DIRECTION('center_axis',(-0.861289491529659,-0.0905598208268723,
0.499979330205146));
#122730=DIRECTION('ref_axis',(0.497139368681318,0.0532207405966013,0.866036951219455));
#122731=DIRECTION('center_axis',(-0.104287292793437,0.994547213842468,-6.79237952684971E-15));
#122732=DIRECTION('ref_axis',(-0.994547213842468,-0.104287292793437,-5.43295081962893E-30));
#122733=DIRECTION('center_axis',(0.994521895368274,0.104528463267647,-1.40045497140052E-16));
#122734=DIRECTION('ref_axis',(-0.104528463267647,0.994521895368274,4.46085091676035E-33));
#122735=DIRECTION('center_axis',(-0.994521895368276,-0.104528463267628,
0.));
#122736=DIRECTION('ref_axis',(0.104528463267628,-0.994521895368276,0.));
#122737=DIRECTION('center_axis',(-2.80862404029962E-16,-1.47193748793057E-17,
-1.));
#122738=DIRECTION('ref_axis',(-1.,-7.33996988677776E-34,2.25664243350207E-16));
#122739=DIRECTION('center_axis',(-0.104769627595152,0.994496518411992,0.));
#122740=DIRECTION('ref_axis',(-0.994496518411992,-0.104769627595152,0.));
#122741=DIRECTION('center_axis',(-0.527021693998977,-0.0553922121162173,
-0.848044713969329));
#122742=DIRECTION('ref_axis',(-0.849348742192414,-1.83506661866328E-16,
0.527832088960271));
#122743=DIRECTION('center_axis',(-0.527021177161337,-0.0553921577943458,
0.848045038708656));
#122744=DIRECTION('ref_axis',(0.849349064867525,1.12341132698979E-15,0.527831569734759));
#122745=DIRECTION('center_axis',(-0.527021723799615,-0.0553922405967594,
-0.84804469358929));
#122746=DIRECTION('ref_axis',(0.843864204095484,0.0841354767076637,-0.529919264233213));
#122747=DIRECTION('center_axis',(-0.527021758969971,-0.0553922189449439,
-0.848044673146736));
#122748=DIRECTION('ref_axis',(-0.849348701629311,-1.08810580052108E-15,
0.527832154231441));
#122749=DIRECTION('center_axis',(0.527021207297265,0.0553921391468907,-0.848045021198559));
#122750=DIRECTION('ref_axis',(-0.842941044393171,-0.0929299148386683,-0.529919264233174));
#122751=DIRECTION('center_axis',(-0.527021232978637,-0.0553921636609804,
0.848045003637562));
#122752=DIRECTION('ref_axis',(0.849349030019363,3.97632889144078E-16,0.527831625809943));
#122753=DIRECTION('center_axis',(-0.104271693993661,0.994548849394384,-1.09530233639679E-15));
#122754=DIRECTION('ref_axis',(-0.994548849394384,-0.104271693993661,-4.95157661577672E-30));
#122755=DIRECTION('center_axis',(-0.994521895368276,-0.104528463267629,
0.));
#122756=DIRECTION('ref_axis',(0.104528463267629,-0.994521895368276,0.));
#122757=DIRECTION('center_axis',(-2.80862404029962E-16,-1.47193748793057E-17,
-1.));
#122758=DIRECTION('ref_axis',(-1.,6.7718648802349E-34,2.40228573745067E-16));
#122759=DIRECTION('center_axis',(-0.104785225574079,0.994494875050339,5.72514616500429E-15));
#122760=DIRECTION('ref_axis',(-0.994494875050339,-0.104785225574079,-6.43259793743591E-30));
#122761=DIRECTION('center_axis',(-0.994521895368274,-0.104528463267647,
1.40045497140052E-16));
#122762=DIRECTION('ref_axis',(0.104528463267647,-0.994521895368274,-2.54421857963839E-30));
#122763=DIRECTION('center_axis',(-0.861277224843639,-0.090493676373255,
-0.50001243634743));
#122764=DIRECTION('ref_axis',(0.497169646238253,0.0532497883205307,-0.866017784403501));
#122765=DIRECTION('center_axis',(0.527021758969985,0.0553922189448812,0.848044673146731));
#122766=DIRECTION('ref_axis',(0.849348701629303,2.79217958474986E-16,-0.527832154231454));
#122767=DIRECTION('center_axis',(0.497265928783528,0.0522647653353818,0.866022511471551));
#122768=DIRECTION('ref_axis',(0.860801807879636,0.0949749838176848,-0.499999999999981));
#122769=DIRECTION('center_axis',(-0.497265943181819,-0.0522647566817781,
-0.86602250372637));
#122770=DIRECTION('ref_axis',(-0.867207748104435,5.13864830604783E-16,0.497946504785037));
#122771=DIRECTION('center_axis',(0.527021723598022,0.0553922406572584,0.84804469371062));
#122772=DIRECTION('ref_axis',(0.842916495800095,0.0931523188259858,-0.529919264233176));
#122773=DIRECTION('center_axis',(0.527021693998996,0.0553922121161724,0.84804471396932));
#122774=DIRECTION('ref_axis',(0.849348742192403,5.99585543773934E-16,-0.527832088960289));
#122775=DIRECTION('center_axis',(-0.994521895368276,-0.104528463267629,
0.));
#122776=DIRECTION('ref_axis',(0.104528463267629,-0.994521895368276,0.));
#122777=DIRECTION('center_axis',(0.994521895368276,0.104528463267628,0.));
#122778=DIRECTION('ref_axis',(-0.104528463267628,0.994521895368276,0.));
#122779=DIRECTION('center_axis',(-0.994521895368274,-0.104528463267647,
1.40045497140052E-16));
#122780=DIRECTION('ref_axis',(0.104528463267647,-0.994521895368274,-2.54421857963839E-30));
#122781=DIRECTION('center_axis',(-0.994521895368276,-0.104528463267629,
-5.43376528903392E-14));
#122782=DIRECTION('ref_axis',(0.104528463267629,-0.994521895368276,3.90011821701468E-29));
#122783=DIRECTION('center_axis',(-0.994521895368274,-0.104528463267647,
1.40045497140052E-16));
#122784=DIRECTION('ref_axis',(0.104528463267647,-0.994521895368274,-2.54421857963839E-30));
#122785=DIRECTION('center_axis',(0.861296695145304,0.090491283002778,-0.499979330205048));
#122786=DIRECTION('ref_axis',(0.497340894868902,0.0513033469999677,0.86603695121952));
#122787=DIRECTION('center_axis',(-0.497266077958585,-0.052264770847387,
0.866022425483288));
#122788=DIRECTION('ref_axis',(0.867207670398075,-3.34654605919539E-16,0.497946640115931));
#122789=DIRECTION('center_axis',(-0.497266086882775,-0.0522647717853675,
0.866022420302451));
#122790=DIRECTION('ref_axis',(-0.104528463267235,0.994521895368317,2.09805925415276E-13));
#122791=DIRECTION('center_axis',(0.500005014359855,-5.28472542476178E-25,
0.866022508723071));
#122792=DIRECTION('ref_axis',(0.,-1.,0.));
#122793=DIRECTION('center_axis',(0.866018223015981,3.00422146885054E-5,
0.500012436347045));
#122794=DIRECTION('ref_axis',(0.50001221743854,-0.000989701280687953,-0.866017784403744));
#122795=DIRECTION('center_axis',(-0.500005023014372,1.99980824065794E-14,
-0.866022503726316));
#122796=DIRECTION('ref_axis',(-0.866022503726316,2.47318747560494E-28,0.500005023014372));
#122797=DIRECTION('center_axis',(-1.,0.,0.));
#122798=DIRECTION('ref_axis',(0.,0.,1.));
#122799=DIRECTION('center_axis',(1.,0.,-1.4081690688991E-16));
#122800=DIRECTION('ref_axis',(-1.40816906889911E-16,0.,-1.));
#122801=DIRECTION('center_axis',(1.,0.,0.));
#122802=DIRECTION('ref_axis',(0.,0.,-1.));
#122803=DIRECTION('center_axis',(1.,0.,-1.4081690688991E-16));
#122804=DIRECTION('ref_axis',(-1.40816906889911E-16,0.,-1.));
#122805=DIRECTION('center_axis',(-1.,0.,0.));
#122806=DIRECTION('ref_axis',(0.,0.,1.));
#122807=DIRECTION('center_axis',(0.52992421326579,0.,-0.848045003637563));
#122808=DIRECTION('ref_axis',(-0.848045003637563,0.,-0.52992421326579));
#122809=DIRECTION('center_axis',(-0.500005158533422,0.,0.866022425483294));
#122810=DIRECTION('ref_axis',(0.866022425483294,0.,0.500005158533421));
#122811=DIRECTION('center_axis',(-0.529924185004363,2.16250770144206E-8,
0.848045021297491));
#122812=DIRECTION('ref_axis',(-0.848037146343328,0.00430950303294841,-0.529919264233217));
#122813=DIRECTION('center_axis',(0.529924157141051,0.,-0.848045038708645));
#122814=DIRECTION('ref_axis',(-0.848045038708645,0.,-0.529924157141051));
#122815=DIRECTION('center_axis',(-0.500005172385336,1.05228546522468E-8,
0.866022417485778));
#122816=DIRECTION('ref_axis',(-0.866013458679382,0.00454855869519104,-0.499999999999971));
#122817=DIRECTION('center_axis',(-0.866037336481608,-3.44576746081222E-5,
0.499979330205271));
#122818=DIRECTION('ref_axis',(0.499979069431786,0.000963977571833242,0.866036951219384));
#122819=DIRECTION('center_axis',(1.,0.,-1.4081690688991E-16));
#122820=DIRECTION('ref_axis',(-1.40816906889911E-16,0.,-1.));
#122821=DIRECTION('center_axis',(-1.,0.,0.));
#122822=DIRECTION('ref_axis',(0.,0.,1.));
#122823=DIRECTION('center_axis',(-0.529924676825566,4.63345850078939E-14,
-0.848044713969328));
#122824=DIRECTION('ref_axis',(-0.848044713969328,6.28460543516088E-28,0.529924676825566));
#122825=DIRECTION('center_axis',(-0.529924157141051,0.,0.848045038708645));
#122826=DIRECTION('ref_axis',(0.848045038708645,0.,0.529924157141051));
#122827=DIRECTION('center_axis',(-0.529924709439991,-2.52115190754827E-8,
-0.848044693589283));
#122828=DIRECTION('ref_axis',(0.848035979777046,-0.004533254694808,-0.529919264233201));
#122829=DIRECTION('center_axis',(-0.529924742154432,-7.52880596504244E-14,
-0.848044673146739));
#122830=DIRECTION('ref_axis',(-0.848044673146739,-1.67508848323945E-27,
0.529924742154432));
#122831=DIRECTION('center_axis',(0.529924185162666,-2.16955825930106E-8,
-0.84804502119857));
#122832=DIRECTION('ref_axis',(-0.848037146343333,-0.00430950303298729,-0.529919264233208));
#122833=DIRECTION('center_axis',(-0.52992421326579,0.,0.848045003637563));
#122834=DIRECTION('ref_axis',(0.848045003637563,0.,0.52992421326579));
#122835=DIRECTION('center_axis',(-1.,0.,0.));
#122836=DIRECTION('ref_axis',(0.,0.,1.));
#122837=DIRECTION('center_axis',(-1.,0.,1.4081690688991E-16));
#122838=DIRECTION('ref_axis',(1.40816906889911E-16,0.,1.));
#122839=DIRECTION('center_axis',(-0.866018223014584,3.00422160359115E-5,
-0.500012436349465));
#122840=DIRECTION('ref_axis',(0.500012217440937,0.000989701331542005,-0.866017784402302));
#122841=DIRECTION('center_axis',(0.529924742154432,0.,0.848044673146739));
#122842=DIRECTION('ref_axis',(0.848044673146739,0.,-0.529924742154432));
#122843=DIRECTION('center_axis',(0.500005009599436,1.01138510236107E-8,
0.866022511471537));
#122844=DIRECTION('ref_axis',(0.866013834616156,0.00447641077665378,-0.49999999999998));
#122845=DIRECTION('center_axis',(-0.50000502301429,0.,-0.866022503726363));
#122846=DIRECTION('ref_axis',(-0.866022503726363,0.,0.50000502301429));
#122847=DIRECTION('center_axis',(0.529924709245824,2.5290276851337E-8,0.848044693710614));
#122848=DIRECTION('ref_axis',(0.84803597977705,0.00453325469478472,-0.529919264233196));
#122849=DIRECTION('center_axis',(0.529924676825566,-2.89534733035821E-14,
0.848044713969328));
#122850=DIRECTION('ref_axis',(0.848044713969328,-3.88919656581317E-28,-0.529924676825566));
#122851=DIRECTION('center_axis',(-1.,0.,0.));
#122852=DIRECTION('ref_axis',(0.,0.,1.));
#122853=DIRECTION('center_axis',(1.,0.,0.));
#122854=DIRECTION('ref_axis',(0.,0.,-1.));
#122855=DIRECTION('center_axis',(-1.,0.,1.4081690688991E-16));
#122856=DIRECTION('ref_axis',(1.40816906889911E-16,0.,1.));
#122857=DIRECTION('center_axis',(-1.,0.,-5.46369598732844E-14));
#122858=DIRECTION('ref_axis',(-5.46369598732844E-14,0.,1.));
#122859=DIRECTION('center_axis',(-1.,0.,1.4081690688991E-16));
#122860=DIRECTION('ref_axis',(1.40816906889911E-16,0.,1.));
#122861=DIRECTION('center_axis',(0.866037336481682,-3.44576746592244E-5,
-0.499979330205142));
#122862=DIRECTION('ref_axis',(0.499979069431655,-0.0009639775757032,0.866036951219455));
#122863=DIRECTION('center_axis',(-0.500005158533445,0.,0.866022425483281));
#122864=DIRECTION('ref_axis',(0.866022425483281,0.,0.500005158533445));
#122865=DIRECTION('center_axis',(-0.500005167507542,-1.62899615243472E-20,
0.866022420302012));
#122866=DIRECTION('ref_axis',(2.517671104983E-12,1.,1.43367382367087E-12));
#122867=DIRECTION('center_axis',(0.497265934578437,-0.0522647557775339,
0.866022508720962));
#122868=DIRECTION('ref_axis',(-0.104528463269674,-0.994521895368061,1.15393259518051E-12));
#122869=DIRECTION('center_axis',(0.861277224842471,-0.0904936763714831,
0.500012436349763));
#122870=DIRECTION('ref_axis',(0.497169646236513,-0.0532497883592382,-0.86601778440212));
#122871=DIRECTION('center_axis',(-0.497265943181921,0.0522647566818165,
-0.866022503726309));
#122872=DIRECTION('ref_axis',(-0.867207748104375,1.06823760381825E-15,0.497946504785141));
#122873=DIRECTION('center_axis',(-0.99452189536827,0.104528463267684,0.));
#122874=DIRECTION('ref_axis',(-0.104528463267684,-0.99452189536827,0.));
#122875=DIRECTION('center_axis',(0.994521895368273,-0.104528463267661,-1.40045497140051E-16));
#122876=DIRECTION('ref_axis',(0.104528463267661,0.994521895368273,1.30294696027314E-33));
#122877=DIRECTION('center_axis',(0.99452189536827,-0.104528463267683,7.13889681646599E-16));
#122878=DIRECTION('ref_axis',(0.104528463267683,0.99452189536827,1.34079853327121E-32));
#122879=DIRECTION('center_axis',(0.994521895368273,-0.104528463267661,-1.40045497140051E-16));
#122880=DIRECTION('ref_axis',(0.104528463267661,0.994521895368273,1.30294696027314E-33));
#122881=DIRECTION('center_axis',(-0.99452189536827,0.104528463267684,0.));
#122882=DIRECTION('ref_axis',(-0.104528463267684,-0.99452189536827,0.));
#122883=DIRECTION('center_axis',(0.527021232978633,-0.055392163661009,-0.848045003637563));
#122884=DIRECTION('ref_axis',(-0.849349030019364,5.85867664728134E-16,-0.52783162580994));
#122885=DIRECTION('center_axis',(-0.497266077958558,0.0522647708474108,
0.866022425483302));
#122886=DIRECTION('ref_axis',(0.86720767039809,-1.24823614703178E-15,0.497946640115905));
#122887=DIRECTION('center_axis',(-0.527021202611211,0.0553921822166726,
0.848045021297518));
#122888=DIRECTION('ref_axis',(-0.842941044394674,0.0929299148248866,-0.529919264233199));
#122889=DIRECTION('center_axis',(0.527021177161334,-0.0553921577943745,
-0.848045038708656));
#122890=DIRECTION('ref_axis',(-0.849349064867527,1.26627050092037E-15,-0.527831569734757));
#122891=DIRECTION('center_axis',(-0.497266090635456,0.052264782753286,0.866022417485762));
#122892=DIRECTION('ref_axis',(-0.860793892491048,0.0950466972078587,-0.499999999999987));
#122893=DIRECTION('center_axis',(-0.861296695145158,0.090491283003084,0.499979330205244));
#122894=DIRECTION('ref_axis',(0.497340894869869,-0.0513033469926123,0.8660369512194));
#122895=DIRECTION('center_axis',(0.104769627595185,0.994496518411988,6.7920332963246E-15));
#122896=DIRECTION('ref_axis',(-0.994496518411988,0.104769627595185,1.05324867106884E-29));
#122897=DIRECTION('center_axis',(0.994521895368273,-0.104528463267661,-1.40045497140051E-16));
#122898=DIRECTION('ref_axis',(0.104528463267661,0.994521895368273,1.30294696027314E-33));
#122899=DIRECTION('center_axis',(-0.99452189536827,0.104528463267682,0.));
#122900=DIRECTION('ref_axis',(-0.104528463267682,-0.99452189536827,0.));
#122901=DIRECTION('center_axis',(-2.80862404029962E-16,1.47193748793076E-17,
-1.));
#122902=DIRECTION('ref_axis',(-1.,7.33996988677776E-34,2.25664243350207E-16));
#122903=DIRECTION('center_axis',(0.104287292793436,0.994547213842468,0.));
#122904=DIRECTION('ref_axis',(-0.994547213842468,0.104287292793436,0.));
#122905=DIRECTION('center_axis',(-0.527021693998993,0.0553922121162014,
-0.84804471396932));
#122906=DIRECTION('ref_axis',(-0.849348742192405,7.73172637784552E-16,0.527832088960287));
#122907=DIRECTION('center_axis',(-0.527021177161343,0.0553921577943754,
0.84804503870865));
#122908=DIRECTION('ref_axis',(0.849349064867521,-6.73775658095366E-16,0.527831569734766));
#122909=DIRECTION('center_axis',(-0.527021729070407,0.0553921904487129,
-0.848044693589277));
#122910=DIRECTION('ref_axis',(0.842916495800679,-0.0931523188207521,-0.529919264233166));
#122911=DIRECTION('center_axis',(-0.527021758969984,0.0553922189448815,
-0.848044673146731));
#122912=DIRECTION('ref_axis',(-0.849348701629303,3.24436902378634E-16,0.527832154231453));
#122913=DIRECTION('center_axis',(0.527021202762083,-0.0553921822962672,
-0.848045021198559));
#122914=DIRECTION('ref_axis',(-0.843841975854018,0.0843581245720705,-0.529919264233212));
#122915=DIRECTION('center_axis',(-0.527021232978546,0.0553921636609998,
0.848045003637618));
#122916=DIRECTION('ref_axis',(0.849349030019419,4.23856781191178E-16,0.527831625809852));
#122917=DIRECTION('center_axis',(0.104785225574091,0.994494875050338,1.06687590778439E-15));
#122918=DIRECTION('ref_axis',(-0.994494875050338,0.104785225574091,-2.00184842661233E-31));
#122919=DIRECTION('center_axis',(-0.99452189536827,0.104528463267683,0.));
#122920=DIRECTION('ref_axis',(-0.104528463267683,-0.99452189536827,0.));
#122921=DIRECTION('center_axis',(-2.80862404029962E-16,1.47193748793076E-17,
-1.));
#122922=DIRECTION('ref_axis',(-1.,-6.7718648802349E-34,2.40228573745067E-16));
#122923=DIRECTION('center_axis',(0.104271693993677,0.994548849394382,1.0953023363959E-15));
#122924=DIRECTION('ref_axis',(-0.994548849394382,0.104271693993677,-2.24841715580815E-30));
#122925=DIRECTION('center_axis',(-0.994521895368273,0.104528463267661,1.40045497140051E-16));
#122926=DIRECTION('ref_axis',(-0.104528463267661,-0.994521895368273,-3.17226103509723E-30));
#122927=DIRECTION('center_axis',(-0.86127094430936,0.0905534316549058,-0.500012436349321));
#122928=DIRECTION('ref_axis',(0.497376550151829,-0.0512812290979085,-0.866017784402418));
#122929=DIRECTION('center_axis',(0.527021758969972,-0.0553922189449264,
0.848044673146736));
#122930=DIRECTION('ref_axis',(0.84934870162931,-1.04254574140673E-15,-0.527832154231442));
#122931=DIRECTION('center_axis',(0.497265930897757,-0.0522647452198303,
0.866022511471551));
#122932=DIRECTION('ref_axis',(0.861737632556863,-0.0860712067727678,-0.499999999999973));
#122933=DIRECTION('center_axis',(-0.497265943181812,0.0522647566818046,
-0.866022503726373));
#122934=DIRECTION('ref_axis',(-0.867207748104439,-1.05899293295569E-16,
0.497946504785031));
#122935=DIRECTION('center_axis',(0.52702172888492,-0.0553921903558326,0.848044693710617));
#122936=DIRECTION('ref_axis',(0.843864204094707,-0.0841354767155294,-0.529919264233202));
#122937=DIRECTION('center_axis',(0.527021693998975,-0.0553922121162288,
0.848044713969329));
#122938=DIRECTION('ref_axis',(0.849348742192415,-2.80634281047211E-16,-0.52783208896027));
#122939=DIRECTION('center_axis',(-0.99452189536827,0.104528463267683,-7.13889681646599E-16));
#122940=DIRECTION('ref_axis',(-0.104528463267683,-0.99452189536827,-1.34079853327121E-32));
#122941=DIRECTION('center_axis',(0.99452189536827,-0.104528463267683,0.));
#122942=DIRECTION('ref_axis',(0.104528463267683,0.99452189536827,0.));
#122943=DIRECTION('center_axis',(-0.994521895368273,0.104528463267661,1.40045497140051E-16));
#122944=DIRECTION('ref_axis',(-0.104528463267661,-0.994521895368273,-3.17226103509723E-30));
#122945=DIRECTION('center_axis',(-0.99452189536827,0.104528463267683,0.));
#122946=DIRECTION('ref_axis',(-0.104528463267683,-0.99452189536827,0.));
#122947=DIRECTION('center_axis',(-0.994521895368273,0.104528463267661,1.40045497140051E-16));
#122948=DIRECTION('ref_axis',(-0.104528463267661,-0.994521895368273,-3.17226103509723E-30));
#122949=DIRECTION('center_axis',(0.861289491529929,-0.0905598208278999,
-0.499979330204495));
#122950=DIRECTION('ref_axis',(0.497139368682485,-0.0532207405793518,0.866036951219846));
#122951=DIRECTION('center_axis',(-0.497266077958593,0.0522647708474152,
0.866022425483281));
#122952=DIRECTION('ref_axis',(0.86720767039807,8.55165079355547E-16,0.497946640115939));
#122953=DIRECTION('center_axis',(-0.497266086886414,0.0522647717857493,
0.866022420300339));
#122954=DIRECTION('ref_axis',(0.104528463264132,0.994521895368643,-2.02812394566828E-12));
#122955=DIRECTION('center_axis',(0.489078705152892,-0.103956887953326,0.866022508721933));
#122956=DIRECTION('ref_axis',(-0.207911690816164,-0.978147600734145,-9.44126668779075E-13));
#122957=DIRECTION('center_axis',(0.847099893161435,-0.180025927304715,0.5000124363493));
#122958=DIRECTION('ref_axis',(0.488879980346119,-0.104926459558925,-0.866017784402381));
#122959=DIRECTION('center_axis',(-0.489078713616374,0.103956889752291,-0.866022503726308));
#122960=DIRECTION('ref_axis',(-0.8707403454847,1.34673219974783E-15,0.491743073916842));
#122961=DIRECTION('center_axis',(-0.978147600733806,0.207911690817757,0.));
#122962=DIRECTION('ref_axis',(-0.207911690817757,-0.978147600733806,0.));
#122963=DIRECTION('center_axis',(0.978147600733804,-0.207911690817766,-1.37739719617121E-16));
#122964=DIRECTION('ref_axis',(0.207911690817766,0.978147600733804,1.60446558522523E-32));
#122965=DIRECTION('center_axis',(0.978147600733806,-0.207911690817757,2.83991567709912E-15));
#122966=DIRECTION('ref_axis',(0.207911690817757,0.978147600733806,3.75217731718872E-32));
#122967=DIRECTION('center_axis',(0.978147600733804,-0.207911690817766,-1.37739719617121E-16));
#122968=DIRECTION('ref_axis',(0.207911690817766,0.978147600733804,3.71870420817402E-33));
#122969=DIRECTION('center_axis',(-0.978147600733806,0.207911690817757,0.));
#122970=DIRECTION('ref_axis',(-0.207911690817757,-0.978147600733806,0.));
#122971=DIRECTION('center_axis',(0.518344097776651,-0.110177439185353,-0.848045003637583));
#122972=DIRECTION('ref_axis',(-0.85323958281187,-2.80350702506811E-15,-0.521519140898037));
#122973=DIRECTION('center_axis',(-0.489078846174,0.103956917928285,0.86602242548329));
#122974=DIRECTION('ref_axis',(0.870740269393777,4.88633091176988E-16,0.4917432086527));
#122975=DIRECTION('center_axis',(-0.518344065636028,0.110177454465083,0.848045021297518));
#122976=DIRECTION('ref_axis',(-0.828609503964381,0.180532167035406,-0.52991926423315));
#122977=DIRECTION('center_axis',(0.518344042878403,-0.110177427516371,-0.848045038708645));
#122978=DIRECTION('ref_axis',(-0.8532396169873,6.46440564947912E-16,-0.521519084984783));
#122979=DIRECTION('center_axis',(-0.489078857536097,0.103956931097731,0.866022417485788));
#122980=DIRECTION('ref_axis',(-0.846143288282855,0.18450348423242,-0.499999999999975));
#122981=DIRECTION('center_axis',(-0.847119506978905,0.180025582247166,0.499979330205145));
#122982=DIRECTION('ref_axis',(0.489253749388084,-0.103008581352267,0.866036951219459));
#122983=DIRECTION('center_axis',(0.208148881407623,0.978097154258592,-1.33600637423501E-14));
#122984=DIRECTION('ref_axis',(-0.978097154258592,0.208148881407623,6.0960315452562E-29));
#122985=DIRECTION('center_axis',(0.978147600733804,-0.207911690817766,-1.37739719617121E-16));
#122986=DIRECTION('ref_axis',(0.207911690817766,0.978147600733804,1.60446558522523E-32));
#122987=DIRECTION('center_axis',(-0.978147600733806,0.20791169081776,0.));
#122988=DIRECTION('ref_axis',(-0.20791169081776,-0.978147600733805,0.));
#122989=DIRECTION('center_axis',(-2.78556626507032E-16,2.92774812072093E-17,
-1.));
#122990=DIRECTION('ref_axis',(-1.,1.56586024251259E-33,2.25664243350207E-16));
#122991=DIRECTION('center_axis',(0.20767448800183,0.978197989689806,0.));
#122992=DIRECTION('ref_axis',(-0.978197989689806,0.20767448800183,0.));
#122993=DIRECTION('center_axis',(-0.518344551206579,0.11017753556484,-0.848044713969322));
#122994=DIRECTION('ref_axis',(-0.853239300541044,-9.36522703165552E-16,
0.521519602711375));
#122995=DIRECTION('center_axis',(-0.518344042878406,0.110177427516371,0.848045038708643));
#122996=DIRECTION('ref_axis',(0.853239616987298,-2.86146343343731E-16,0.521519084984786));
#122997=DIRECTION('center_axis',(-0.518344588350167,0.110177517684659,-0.848044693589284));
#122998=DIRECTION('ref_axis',(0.828561842306931,-0.180750786630268,-0.529919264233226));
#122999=DIRECTION('center_axis',(-0.518344615107843,0.110177549147442,-0.848044673146742));
#123000=DIRECTION('ref_axis',(-0.853239260760972,-3.62990359272678E-15,
0.521519667794101));
#123001=DIRECTION('center_axis',(0.51834406577791,-0.110177454559223,-0.848045021198566));
#123002=DIRECTION('ref_axis',(-0.830401496089648,0.172101506927106,-0.529919264233236));
#123003=DIRECTION('center_axis',(-0.518344097776628,0.110177439185349,0.848045003637597));
#123004=DIRECTION('ref_axis',(0.853239582811884,-1.82149902462599E-16,0.521519140898014));
#123005=DIRECTION('center_axis',(0.208164222161113,0.978093889466681,-1.13734602532708E-14));
#123006=DIRECTION('ref_axis',(-0.978093889466681,0.208164222161113,-1.1232129081755E-29));
#123007=DIRECTION('center_axis',(-0.978147600733806,0.207911690817757,-5.67983135419856E-15));
#123008=DIRECTION('ref_axis',(-0.207911690817757,-0.978147600733806,1.30668494926232E-31));
#123009=DIRECTION('center_axis',(-2.78556626507032E-16,2.92774812072093E-17,
-1.));
#123010=DIRECTION('ref_axis',(-1.,-1.27623607358273E-33,2.40228573745067E-16));
#123011=DIRECTION('center_axis',(0.207659145615657,0.978201246800563,2.0156211610367E-15));
#123012=DIRECTION('ref_axis',(-0.978201246800563,0.207659145615657,-8.6231864451917E-30));
#123013=DIRECTION('center_axis',(-0.978147600733804,0.207911690817766,1.37739719617121E-16));
#123014=DIRECTION('ref_axis',(-0.207911690817766,-0.978147600733804,1.32119636604405E-30));
#123015=DIRECTION('center_axis',(-0.847087400905852,0.180084698747157,-0.500012436349051));
#123016=DIRECTION('ref_axis',(0.489291521294912,-0.102990311618894,-0.86601778440258));
#123017=DIRECTION('center_axis',(0.518344615107832,-0.110177549147519,0.848044673146739));
#123018=DIRECTION('ref_axis',(0.853239260760976,2.80072453551802E-15,-0.521519667794095));
#123019=DIRECTION('center_axis',(0.489078702597842,-0.103956877068183,0.866022511471522));
#123020=DIRECTION('ref_axis',(0.848020052665161,-0.175675810166694,-0.500000000000054));
#123021=DIRECTION('center_axis',(-0.489078713616299,0.103956889752277,-0.866022503726352));
#123022=DIRECTION('ref_axis',(-0.870740345484743,-2.29938292486793E-15,
0.491743073916766));
#123023=DIRECTION('center_axis',(0.518344588177269,-0.110177517564182,0.848044693710616));
#123024=DIRECTION('ref_axis',(0.830446875605224,-0.171882402217535,-0.529919264233195));
#123025=DIRECTION('center_axis',(0.518344551206566,-0.110177535564839,0.84804471396933));
#123026=DIRECTION('ref_axis',(0.853239300541052,2.40506994729313E-15,-0.521519602711362));
#123027=DIRECTION('center_axis',(-0.978147600733806,0.207911690817757,-2.83991567709928E-15));
#123028=DIRECTION('ref_axis',(-0.207911690817757,-0.978147600733806,6.5334247463116E-32));
#123029=DIRECTION('center_axis',(0.978147600733807,-0.207911690817751,0.));
#123030=DIRECTION('ref_axis',(0.207911690817751,0.978147600733807,0.));
#123031=DIRECTION('center_axis',(-0.978147600733804,0.207911690817766,1.37739719617121E-16));
#123032=DIRECTION('ref_axis',(-0.207911690817766,-0.978147600733804,1.32119636604405E-30));
#123033=DIRECTION('center_axis',(-0.978147600733806,0.207911690817757,-5.91228425656406E-14));
#123034=DIRECTION('ref_axis',(-0.207911690817757,-0.978147600733806,-1.10389829321544E-30));
#123035=DIRECTION('center_axis',(-0.978147600733804,0.207911690817766,1.37739719617121E-16));
#123036=DIRECTION('ref_axis',(-0.207911690817766,-0.978147600733804,1.32119636604405E-30));
#123037=DIRECTION('center_axis',(0.847105178672255,-0.180092991631758,-0.499979330204529));
#123038=DIRECTION('ref_axis',(0.488852904980983,-0.104894406016243,0.866036951219839));
#123039=DIRECTION('center_axis',(-0.489078846174022,0.103956917928291,0.866022425483277));
#123040=DIRECTION('ref_axis',(0.870740269393764,-1.77516479390848E-15,0.491743208652722));
#123041=DIRECTION('center_axis',(-0.489078854950438,0.103956919793789,0.866022420302937));
#123042=DIRECTION('ref_axis',(0.207911690821673,0.978147600732974,2.30786517957212E-12));
#123043=DIRECTION('center_axis',(0.475533027088914,-0.154510046710454,0.866022508722024));
#123044=DIRECTION('ref_axis',(-0.309016994376972,-0.951056516294496,1.18890024960415E-12));
#123045=DIRECTION('center_axis',(0.823641557784546,-0.267585776505932,0.500012436347302));
#123046=DIRECTION('ref_axis',(0.475234043107506,-0.155453534435146,-0.866017784403596));
#123047=DIRECTION('center_axis',(-0.47553303531813,0.154510049384315,-0.866022503726308));
#123048=DIRECTION('ref_axis',(-0.876548788012439,-2.73579469640639E-15,
0.48131301897406));
#123049=DIRECTION('center_axis',(-0.951056516295146,0.309016994374972,0.));
#123050=DIRECTION('ref_axis',(-0.309016994374972,-0.951056516295146,0.));
#123051=DIRECTION('center_axis',(0.951056516295151,-0.309016994374955,-1.33924836902177E-16));
#123052=DIRECTION('ref_axis',(0.309016994374955,0.951056516295151,-1.26216548479895E-32));
#123053=DIRECTION('center_axis',(0.951056516295148,-0.309016994374964,0.));
#123054=DIRECTION('ref_axis',(0.309016994374964,0.951056516295148,0.));
#123055=DIRECTION('center_axis',(0.951056516295151,-0.309016994374955,-1.33924836902177E-16));
#123056=DIRECTION('ref_axis',(0.309016994374955,0.951056516295151,-2.95703203911168E-34));
#123057=DIRECTION('center_axis',(-0.951056516295151,0.309016994374956,0.));
#123058=DIRECTION('ref_axis',(-0.309016994374956,-0.951056516295151,0.));
#123059=DIRECTION('center_axis',(0.503987876168974,-0.1637555876299,-0.848045003637586));
#123060=DIRECTION('ref_axis',(-0.859649462041495,-1.25677763959017E-15,
-0.510884333691853));
#123061=DIRECTION('center_axis',(-0.475533164204393,0.154510091261982,0.866022425483296));
#123062=DIRECTION('ref_axis',(0.876548714628846,-1.09074871697088E-16,0.481313152617419));
#123063=DIRECTION('center_axis',(-0.503987842609045,0.163755599460945,0.848045021297494));
#123064=DIRECTION('ref_axis',(-0.805199544418188,0.266156471015187,-0.529919264233227));
#123065=DIRECTION('center_axis',(0.503987822791202,-0.163755570286411,-0.848045038708651));
#123066=DIRECTION('ref_axis',(-0.859649495083704,7.85201449699707E-16,-0.510884278092732));
#123067=DIRECTION('center_axis',(-0.475533174127523,0.154510105547485,0.866022417485776));
#123068=DIRECTION('ref_axis',(-0.822222161142181,0.271938812468327,-0.499999999999997));
#123069=DIRECTION('center_axis',(-0.823661100222764,0.267587483540024,0.499979330205303));
#123070=DIRECTION('ref_axis',(0.475806237442976,-0.153585232144924,0.866036951219374));
#123071=DIRECTION('center_axis',(0.309247612517411,0.950981553003149,2.59793704758334E-14));
#123072=DIRECTION('ref_axis',(-0.950981553003149,0.309247612517411,-2.01038495813744E-28));
#123073=DIRECTION('center_axis',(0.951056516295151,-0.309016994374955,-1.33924836902177E-16));
#123074=DIRECTION('ref_axis',(0.309016994374955,0.951056516295151,-1.26216548479895E-32));
#123075=DIRECTION('center_axis',(-0.951056516295151,0.309016994374956,0.));
#123076=DIRECTION('ref_axis',(-0.309016994374956,-0.951056516295151,0.));
#123077=DIRECTION('center_axis',(-2.74741743792087E-16,4.3514817324298E-17,
-1.));
#123078=DIRECTION('ref_axis',(-1.,-2.34879036376888E-33,2.25664243350207E-16));
#123079=DIRECTION('center_axis',(0.308786358060997,0.951131423661013,0.));
#123080=DIRECTION('ref_axis',(-0.951131423661013,0.308786358060997,0.));
#123081=DIRECTION('center_axis',(-0.503988317040562,0.163755730877734,-0.848044713969329));
#123082=DIRECTION('ref_axis',(-0.859649189130478,3.14369996253285E-15,0.510884792910605));
#123083=DIRECTION('center_axis',(-0.503987822791237,0.163755570286422,0.848045038708627));
#123084=DIRECTION('ref_axis',(0.859649495083682,-1.36481806660529E-15,0.510884278092769));
#123085=DIRECTION('center_axis',(-0.503988355851142,0.163755716973661,-0.848044693589262));
#123086=DIRECTION('ref_axis',(0.805129291876029,-0.266368911019599,-0.529919264233182));
#123087=DIRECTION('center_axis',(-0.503988379172014,0.163755751065422,-0.848044673146743));
#123088=DIRECTION('ref_axis',(-0.859649150669462,5.07104693475844E-15,0.510884857627698));
#123089=DIRECTION('center_axis',(0.50398784273828,-0.163755599575522,-0.848045021198566));
#123090=DIRECTION('ref_axis',(-0.807862963766318,0.257959309134735,-0.529919264233177));
#123091=DIRECTION('center_axis',(-0.503987876168969,0.163755587629899,0.848045003637589));
#123092=DIRECTION('ref_axis',(0.859649462041497,4.5006472016428E-16,0.510884333691849));
#123093=DIRECTION('center_axis',(0.309262527968972,0.95097670255072,0.));
#123094=DIRECTION('ref_axis',(-0.95097670255072,0.309262527968972,0.));
#123095=DIRECTION('center_axis',(-0.951056516295148,0.309016994374964,0.));
#123096=DIRECTION('ref_axis',(-0.309016994374964,-0.951056516295148,0.));
#123097=DIRECTION('center_axis',(-2.74741743792087E-16,4.3514817324298E-17,
-1.));
#123098=DIRECTION('ref_axis',(-1.,-1.71901185421347E-33,2.40228573745067E-16));
#123099=DIRECTION('center_axis',(0.308771440182806,0.951136266645025,0.));
#123100=DIRECTION('ref_axis',(-0.951136266645025,0.308771440182806,0.));
#123101=DIRECTION('center_axis',(-0.951056516295151,0.309016994374955,1.33924836902177E-16));
#123102=DIRECTION('ref_axis',(-0.309016994374955,-0.951056516295151,-1.27877458305741E-30));
#123103=DIRECTION('center_axis',(-0.823622990672807,0.267642920195442,-0.500012436349775));
#123104=DIRECTION('ref_axis',(0.475845712143356,-0.153571010721301,-0.866017784402157));
#123105=DIRECTION('center_axis',(0.503988379171984,-0.163755751065568,0.848044673146732));
#123106=DIRECTION('ref_axis',(0.859649150669473,3.71306128357102E-15,-0.510884857627679));
#123107=DIRECTION('center_axis',(0.475533025685365,-0.154510035619035,0.86602251147157));
#123108=DIRECTION('ref_axis',(0.825011387614939,-0.263355672628674,-0.499999999999972));
#123109=DIRECTION('center_axis',(-0.475533035318107,0.15451004938428,-0.866022503726327));
#123110=DIRECTION('ref_axis',(-0.876548788012453,1.8240586479188E-15,0.481313018974034));
#123111=DIRECTION('center_axis',(0.503988355690598,-0.163755716839192,0.848044693710638));
#123112=DIRECTION('ref_axis',(0.80793099735983,-0.257746148176285,-0.529919264233183));
#123113=DIRECTION('center_axis',(0.503988317040544,-0.163755730877805,0.848044713969326));
#123114=DIRECTION('ref_axis',(0.859649189130486,1.98206584939501E-15,-0.510884792910592));
#123115=DIRECTION('center_axis',(-0.951056516295148,0.309016994374964,0.));
#123116=DIRECTION('ref_axis',(-0.309016994374964,-0.951056516295148,0.));
#123117=DIRECTION('center_axis',(0.951056516295148,-0.309016994374964,0.));
#123118=DIRECTION('ref_axis',(0.309016994374964,0.951056516295148,0.));
#123119=DIRECTION('center_axis',(-0.951056516295151,0.309016994374955,1.33924836902177E-16));
#123120=DIRECTION('ref_axis',(-0.309016994374955,-0.951056516295151,-1.27877458305741E-30));
#123121=DIRECTION('center_axis',(-0.951056516295148,0.309016994374964,-8.44187456091391E-15));
#123122=DIRECTION('ref_axis',(-0.309016994374964,-0.951056516295148,7.16904701312154E-29));
#123123=DIRECTION('center_axis',(-0.951056516295151,0.309016994374955,1.33924836902177E-16));
#123124=DIRECTION('ref_axis',(-0.309016994374955,-0.951056516295151,-1.27877458305741E-30));
#123125=DIRECTION('center_axis',(0.823639804208732,-0.26765302593154,-0.499979330205452));
#123126=DIRECTION('ref_axis',(0.475210466541805,-0.155418826439845,0.866036951219277));
#123127=DIRECTION('center_axis',(-0.47553316420442,0.154510091261982,0.866022425483281));
#123128=DIRECTION('ref_axis',(0.876548714628831,4.67206082329057E-15,0.481313152617445));
#123129=DIRECTION('center_axis',(-0.475533172734512,0.154510094033577,0.866022420304916));
#123130=DIRECTION('ref_axis',(0.309016994377262,0.951056516294402,1.39870616943622E-12));
#123131=DIRECTION('center_axis',(0.456777309663209,-0.203370361060108,0.86602250872545));
#123132=DIRECTION('ref_axis',(-0.406736643086926,-0.913545457637647,7.02849853442907E-12));
#123133=DIRECTION('center_axis',(0.79115923314091,-0.352213899940629,0.500012436349837));
#123134=DIRECTION('ref_axis',(0.456381342241232,-0.204277427909412,-0.866017784402149));
#123135=DIRECTION('center_axis',(-0.456777317573273,0.203370364581912,-0.86602250372631));
#123136=DIRECTION('ref_axis',(-0.884507036382098,5.88362210846088E-15,0.466526850878444));
#123137=DIRECTION('center_axis',(-0.913545457642594,0.406736643075817,0.));
#123138=DIRECTION('ref_axis',(-0.406736643075817,-0.913545457642593,0.));
#123139=DIRECTION('center_axis',(0.913545457642598,-0.406736643075807,-1.28642645648558E-16));
#123140=DIRECTION('ref_axis',(0.406736643075807,0.913545457642598,-3.77717422672452E-33));
#123141=DIRECTION('center_axis',(0.913545457642598,-0.406736643075807,0.));
#123142=DIRECTION('ref_axis',(0.406736643075807,0.913545457642598,0.));
#123143=DIRECTION('center_axis',(0.913545457642598,-0.406736643075807,-1.28642645648558E-16));
#123144=DIRECTION('ref_axis',(0.406736643075807,0.913545457642598,-3.77717422672452E-33));
#123145=DIRECTION('center_axis',(-0.913545457642594,0.406736643075817,0.));
#123146=DIRECTION('ref_axis',(-0.406736643075817,-0.913545457642593,0.));
#123147=DIRECTION('center_axis',(0.484109857923749,-0.215539595588297,-0.84804500363759));
#123148=DIRECTION('ref_axis',(-0.868458021516007,5.90166044795577E-15,-0.495762710239992));
#123149=DIRECTION('center_axis',(-0.456777441376078,0.203370419702503,0.866022425483285));
#123150=DIRECTION('ref_axis',(0.884506966812054,-7.65140401810272E-16,0.466526982779067));
#123151=DIRECTION('center_axis',(-0.484109823308551,0.215539603851996,0.848045021297506));
#123152=DIRECTION('ref_axis',(-0.772967650156497,0.348864709029283,-0.529919264233201));
#123153=DIRECTION('center_axis',(0.484109806651292,-0.215539572760328,-0.848045038708643));
#123154=DIRECTION('ref_axis',(-0.868458052949955,-2.13353959478262E-15,
-0.495762655175209));
#123155=DIRECTION('center_axis',(-0.456777449755519,0.203370434938186,0.86602241748577));
#123156=DIRECTION('ref_axis',(-0.789292595945392,0.356394722163228,-0.499999999999979));
#123157=DIRECTION('center_axis',(-0.791178490090539,0.352217640366771,0.499979330205279));
#123158=DIRECTION('ref_axis',(0.457145692798399,-0.202479170974491,0.866036951219378));
#123159=DIRECTION('center_axis',(0.406958162070226,0.913446798847324,0.));
#123160=DIRECTION('ref_axis',(-0.913446798847324,0.406958162070226,0.));
#123161=DIRECTION('center_axis',(0.913545457642598,-0.406736643075807,-1.28642645648558E-16));
#123162=DIRECTION('ref_axis',(0.406736643075807,0.913545457642598,-3.77717422672452E-33));
#123163=DIRECTION('center_axis',(-0.913545457642603,0.406736643075797,0.));
#123164=DIRECTION('ref_axis',(-0.406736643075797,-0.913545457642603,0.));
#123165=DIRECTION('center_axis',(-2.69459552538469E-16,5.72753959967207E-17,
-1.));
#123166=DIRECTION('ref_axis',(-1.,-2.74025542439703E-33,2.25664243350207E-16));
#123167=DIRECTION('center_axis',(0.406515100163544,0.913644062717546,0.));
#123168=DIRECTION('ref_axis',(-0.913644062717546,0.406515100163544,0.));
#123169=DIRECTION('center_axis',(-0.484110281406756,0.21553978413508,-0.848044713969302));
#123170=DIRECTION('ref_axis',(-0.868457761888264,2.25907686083393E-15,0.495763165045597));
#123171=DIRECTION('center_axis',(-0.48410980665131,0.215539572760337,0.84804503870863));
#123172=DIRECTION('ref_axis',(0.868458052949943,-2.95523665556292E-15,0.49576265517523));
#123173=DIRECTION('center_axis',(-0.484110321457893,0.215539774364283,-0.848044693589277));
#123174=DIRECTION('ref_axis',(0.772875576437821,-0.349068641875063,-0.529919264233152));
#123175=DIRECTION('center_axis',(-0.484110341087621,0.215539810706662,-0.848044673146742));
#123176=DIRECTION('ref_axis',(-0.868457725299266,2.47979274693718E-15,0.495763229140711));
#123177=DIRECTION('center_axis',(0.484109823426302,-0.215539603976822,-0.848045021198562));
#123178=DIRECTION('ref_axis',(-0.776473315751079,0.340990855186838,-0.529919264233217));
#123179=DIRECTION('center_axis',(-0.484109857923765,0.215539595588304,0.84804500363758));
#123180=DIRECTION('ref_axis',(0.868458021515998,-1.76836178502353E-15,0.495762710240009));
#123181=DIRECTION('center_axis',(0.406972488803041,0.913440415876952,0.));
#123182=DIRECTION('ref_axis',(-0.913440415876952,0.406972488803041,0.));
#123183=DIRECTION('center_axis',(-0.913545457642598,0.406736643075807,0.));
#123184=DIRECTION('ref_axis',(-0.406736643075807,-0.913545457642598,0.));
#123185=DIRECTION('center_axis',(-2.69459552538469E-16,5.72753959967207E-17,
-1.));
#123186=DIRECTION('ref_axis',(-1.,-1.97946819576097E-33,2.40228573745067E-16));
#123187=DIRECTION('center_axis',(0.40650077023674,0.913650438514062,0.));
#123188=DIRECTION('ref_axis',(-0.913650438514062,0.40650077023674,0.));
#123189=DIRECTION('center_axis',(-0.913545457642598,0.406736643075807,1.28642645648558E-16));
#123190=DIRECTION('ref_axis',(-0.406736643075807,-0.913545457642598,5.69448373698529E-32));
#123191=DIRECTION('center_axis',(-0.791134794599912,0.352268789802041,-0.500012436350098));
#123192=DIRECTION('ref_axis',(0.45718643779245,-0.202469153695468,-0.866017784401967));
#123193=DIRECTION('center_axis',(0.484110341087585,-0.215539810706754,0.848044673146739));
#123194=DIRECTION('ref_axis',(0.868457725299281,1.08514503248968E-15,-0.495763229140683));
#123195=DIRECTION('center_axis',(0.456777309429512,-0.203370349891223,0.866022511471531));
#123196=DIRECTION('ref_axis',(0.792963725156405,-0.348150155229116,-0.50000000000002));
#123197=DIRECTION('center_axis',(-0.456777317573209,0.203370364581883,-0.86602250372635));
#123198=DIRECTION('ref_axis',(-0.884507036382135,-3.12434821125521E-15,
0.466526850878375));
#123199=DIRECTION('center_axis',(0.484110321310578,-0.215539774217795,0.848044693710603));
#123200=DIRECTION('ref_axis',(0.776563258038879,-0.340785973388812,-0.529919264233223));
#123201=DIRECTION('center_axis',(0.484110281406699,-0.215539784135105,0.848044713969328));
#123202=DIRECTION('ref_axis',(0.868457761888295,1.70886789336824E-17,-0.495763165045542));
#123203=DIRECTION('center_axis',(-0.913545457642598,0.406736643075807,0.));
#123204=DIRECTION('ref_axis',(-0.406736643075807,-0.913545457642598,0.));
#123205=DIRECTION('center_axis',(0.913545457642598,-0.406736643075807,0.));
#123206=DIRECTION('ref_axis',(0.406736643075807,0.913545457642598,0.));
#123207=DIRECTION('center_axis',(-0.913545457642598,0.406736643075807,1.28642645648558E-16));
#123208=DIRECTION('ref_axis',(-0.406736643075807,-0.913545457642598,5.69448373698529E-32));
#123209=DIRECTION('center_axis',(-0.913545457642598,0.406736643075807,-4.99133465116398E-14));
#123210=DIRECTION('ref_axis',(-0.406736643075807,-0.913545457642598,-2.82923979546378E-31));
#123211=DIRECTION('center_axis',(-0.913545457642598,0.406736643075807,1.28642645648558E-16));
#123212=DIRECTION('ref_axis',(-0.406736643075807,-0.913545457642598,5.69448373698529E-32));
#123213=DIRECTION('center_axis',(0.791150459692854,-0.352280597671101,-0.499979330205038));
#123214=DIRECTION('ref_axis',(0.456361522796786,-0.204240445634527,0.866036951219524));
#123215=DIRECTION('center_axis',(-0.456777441376069,0.203370419702468,0.866022425483298));
#123216=DIRECTION('ref_axis',(0.884506966812062,6.03592299906791E-15,0.466526982779053));
#123217=DIRECTION('center_axis',(-0.45677744957756,0.203370423354032,0.866022420299972));
#123218=DIRECTION('ref_axis',(0.406736643068276,0.913545457645951,-4.75560097597516E-12));
#123219=DIRECTION('center_axis',(0.433017044454879,-0.250002507179727,0.866022508723308));
#123220=DIRECTION('ref_axis',(-0.499999999994351,-0.8660254037877,-3.77650667513754E-12));
#123221=DIRECTION('center_axis',(0.750008802379408,-0.432983094185632,0.50001243634818));
#123222=DIRECTION('ref_axis',(0.432528431864326,-0.250863215172243,-0.866017784403087));
#123223=DIRECTION('center_axis',(-0.433017051950279,0.250002511507198,-0.866022503726308));
#123224=DIRECTION('ref_axis',(-0.894424794863783,-6.20270810435665E-16,
0.447218387740127));
#123225=DIRECTION('center_axis',(-0.86602540378444,0.499999999999998,0.));
#123226=DIRECTION('ref_axis',(-0.499999999999998,-0.86602540378444,0.));
#123227=DIRECTION('center_axis',(0.866025403784435,-0.500000000000007,-1.2195101864901E-16));
#123228=DIRECTION('ref_axis',(0.500000000000007,0.866025403784434,1.37857749616202E-32));
#123229=DIRECTION('center_axis',(0.866025403784433,-0.50000000000001,-1.36592399683214E-14));
#123230=DIRECTION('ref_axis',(0.50000000000001,0.866025403784433,-1.33215113601878E-31));
#123231=DIRECTION('center_axis',(0.866025403784435,-0.500000000000007,-1.2195101864901E-16));
#123232=DIRECTION('ref_axis',(0.500000000000007,0.866025403784434,1.37857749616202E-32));
#123233=DIRECTION('center_axis',(-0.866025403784433,0.50000000000001,0.));
#123234=DIRECTION('ref_axis',(-0.50000000000001,-0.866025403784433,0.));
#123235=DIRECTION('center_axis',(0.458927830768604,-0.264962106632863,-0.848045003637601));
#123236=DIRECTION('ref_axis',(-0.879478602053344,3.64727084574667E-15,-0.475938429348057));
#123237=DIRECTION('center_axis',(-0.433017169313214,0.25000257926672,0.866022425483289));
#123238=DIRECTION('ref_axis',(0.894424730216418,3.37693802438162E-15,0.447218517033103));
#123239=DIRECTION('center_axis',(-0.45892779548191,0.264962111228503,0.848045021297483));
#123240=DIRECTION('ref_axis',(-0.732266960577926,0.427750712261754,-0.529919264233269));
#123241=DIRECTION('center_axis',(0.45892778216323,-0.264962078570538,-0.848045038708628));
#123242=DIRECTION('ref_axis',(-0.879478631391236,-7.35193596082728E-15,
-0.475938375135057));
#123243=DIRECTION('center_axis',(-0.433017176051311,0.250002595299908,0.866022417485747));
#123244=DIRECTION('ref_axis',(-0.747715375893068,0.436945896711557,-0.500000000000021));
#123245=DIRECTION('center_axis',(-0.750027562856218,0.432988827019233,0.499979330205231));
#123246=DIRECTION('ref_axis',(0.433476564272144,-0.249154705653748,0.866036951219411));
#123247=DIRECTION('center_axis',(0.500209992837911,0.865904130412309,0.));
#123248=DIRECTION('ref_axis',(-0.865904130412309,0.500209992837911,0.));
#123249=DIRECTION('center_axis',(0.866025403784435,-0.500000000000007,-1.2195101864901E-16));
#123250=DIRECTION('ref_axis',(0.500000000000007,0.866025403784434,1.37857749616202E-32));
#123251=DIRECTION('center_axis',(-0.86602540378444,0.499999999999998,0.));
#123252=DIRECTION('ref_axis',(-0.499999999999998,-0.86602540378444,0.));
#123253=DIRECTION('center_axis',(-2.6276792553892E-16,7.04084534449562E-17,
-1.));
#123254=DIRECTION('ref_axis',(-1.,-2.9359879547111E-33,2.25664243350207E-16));
#123255=DIRECTION('center_axis',(0.499789977759954,0.866146626230631,0.));
#123256=DIRECTION('ref_axis',(-0.866146626230631,0.499789977759954,0.));
#123257=DIRECTION('center_axis',(-0.458928232223265,0.264962338412774,-0.848044713969295));
#123258=DIRECTION('ref_axis',(-0.879478359737711,3.22745562485081E-15,0.475938877118758));
#123259=DIRECTION('center_axis',(-0.458927782163224,0.264962078570543,0.84804503870863));
#123260=DIRECTION('ref_axis',(0.879478631391239,5.78561883712524E-15,0.475938375135052));
#123261=DIRECTION('center_axis',(-0.458928273071634,0.264962332890014,-0.8480446935893));
#123262=DIRECTION('ref_axis',(0.732154074467011,-0.427943903608719,-0.529919264233229));
#123263=DIRECTION('center_axis',(-0.458928288799681,0.264962371077192,-0.848044673146733));
#123264=DIRECTION('ref_axis',(-0.879478325588497,-1.70584345960497E-15,
0.475938940222434));
#123265=DIRECTION('center_axis',(0.458927795584395,-0.264962111367593,-0.848045021198565));
#123266=DIRECTION('ref_axis',(-0.736576463592187,0.420286434085738,-0.529919264233262));
#123267=DIRECTION('center_axis',(-0.458927830768623,0.264962106632883,0.848045003637585));
#123268=DIRECTION('ref_axis',(0.879478602053333,2.80327366676551E-15,0.475938429348078));
#123269=DIRECTION('center_axis',(0.500223573885336,0.865896284857131,1.99792452361211E-14));
#123270=DIRECTION('ref_axis',(-0.865896284857131,0.500223573885336,1.39216074893221E-28));
#123271=DIRECTION('center_axis',(-0.866025403784433,0.50000000000001,0.));
#123272=DIRECTION('ref_axis',(-0.50000000000001,-0.866025403784433,0.));
#123273=DIRECTION('center_axis',(-2.6276792553892E-16,7.04084534449562E-17,
-1.));
#123274=DIRECTION('ref_axis',(-1.,-1.97946819576097E-33,2.40228573745067E-16));
#123275=DIRECTION('center_axis',(0.499776392786197,0.866154464985095,-3.64423934454608E-15));
#123276=DIRECTION('ref_axis',(-0.866154464985095,0.499776392786197,-1.32824799399631E-29));
#123277=DIRECTION('center_axis',(-0.866025403784435,0.500000000000007,1.2195101864901E-16));
#123278=DIRECTION('ref_axis',(-0.500000000000007,-0.866025403784435,-3.8972730010601E-31));
#123279=DIRECTION('center_axis',(-0.749978760164197,0.433035128829165,-0.50001243634782));
#123280=DIRECTION('ref_axis',(-0.433518133165547,0.249149002233455,0.866017784403261));
#123281=DIRECTION('center_axis',(0.458928288799652,-0.264962371077221,0.848044673146739));
#123282=DIRECTION('ref_axis',(0.87947832558851,-5.62014896054226E-15,-0.475938940222411));
#123283=DIRECTION('center_axis',(0.433017045388115,-0.250002496043341,0.866022511471524));
#123284=DIRECTION('ref_axis',(0.752228186189541,-0.429130231866715,-0.500000000000012));
#123285=DIRECTION('center_axis',(-0.433017051950174,0.250002511507138,-0.866022503726378));
#123286=DIRECTION('ref_axis',(-0.894424794863841,8.78579593512627E-16,0.447218387740013));
#123287=DIRECTION('center_axis',(0.458928272946657,-0.264962332718179,0.848044693710621));
#123288=DIRECTION('ref_axis',(0.736687329165484,-0.420092076147145,-0.529919264233155));
#123289=DIRECTION('center_axis',(0.458928232223185,-0.264962338412827,0.848044713969322));
#123290=DIRECTION('ref_axis',(0.879478359737754,5.93852501903154E-15,-0.47593887711868));
#123291=DIRECTION('center_axis',(-0.866025403784433,0.50000000000001,0.));
#123292=DIRECTION('ref_axis',(-0.50000000000001,-0.866025403784433,0.));
#123293=DIRECTION('center_axis',(0.866025403784433,-0.50000000000001,0.));
#123294=DIRECTION('ref_axis',(0.50000000000001,0.866025403784433,0.));
#123295=DIRECTION('center_axis',(-0.866025403784435,0.500000000000007,1.2195101864901E-16));
#123296=DIRECTION('ref_axis',(-0.500000000000007,-0.866025403784435,-3.8972730010601E-31));
#123297=DIRECTION('center_axis',(-0.866025403784433,0.50000000000001,-4.09777199049641E-14));
#123298=DIRECTION('ref_axis',(-0.50000000000001,-0.866025403784433,-3.99645340805632E-31));
#123299=DIRECTION('center_axis',(-0.866025403784435,0.500000000000007,1.2195101864901E-16));
#123300=DIRECTION('ref_axis',(-0.500000000000007,-0.866025403784435,-3.8972730010601E-31));
#123301=DIRECTION('center_axis',(0.749993105181602,-0.433048509462509,-0.499979330205118));
#123302=DIRECTION('ref_axis',(-0.43251258669988,0.250824363786029,-0.866036951219469));
#123303=DIRECTION('center_axis',(-0.433017169313192,0.250002579266708,0.866022425483304));
#123304=DIRECTION('ref_axis',(0.894424730216429,-3.15083324732399E-15,0.44721851703308));
#123305=DIRECTION('center_axis',(-0.433017177084066,0.250002583753203,0.866022420302656));
#123306=DIRECTION('ref_axis',(0.5000000000025,0.866025403782995,1.71341505755983E-12));
#123307=DIRECTION('center_axis',(0.404512553894632,-0.293895573516493,0.866022508719637));
#123308=DIRECTION('ref_axis',(-0.587785252288474,-0.809016994377853,-2.8323800063508E-12));
#123309=DIRECTION('center_axis',(0.700641118228508,-0.509008435042022,0.500012436348915));
#123310=DIRECTION('ref_axis',(0.403936649436713,-0.294700492602699,-0.866017784402589));
#123311=DIRECTION('center_axis',(-0.404512560891457,0.293895578600019,-0.866022503726315));
#123312=DIRECTION('ref_axis',(-0.906035256115487,-3.15407140147818E-15,
0.423202214875754));
#123313=DIRECTION('center_axis',(-0.80901699437495,0.58778525229247,-3.2114799243612E-14));
#123314=DIRECTION('ref_axis',(-0.58778525229247,-0.80901699437495,4.13565546558353E-30));
#123315=DIRECTION('center_axis',(0.809016994374943,-0.58778525229248,-1.13923270769252E-16));
#123316=DIRECTION('ref_axis',(0.58778525229248,0.809016994374943,4.71515639841956E-33));
#123317=DIRECTION('center_axis',(0.809016994374931,-0.587785252292496,-4.42022290584682E-14));
#123318=DIRECTION('ref_axis',(0.587785252292496,0.809016994374931,4.35974171970421E-30));
#123319=DIRECTION('center_axis',(0.809016994374943,-0.58778525229248,-1.13923270769252E-16));
#123320=DIRECTION('ref_axis',(0.58778525229248,0.809016994374943,4.71515639841956E-33));
#123321=DIRECTION('center_axis',(-0.80901699437495,0.58778525229247,0.));
#123322=DIRECTION('ref_axis',(-0.58778525229247,-0.80901699437495,0.));
#123323=DIRECTION('center_axis',(0.428717694262752,-0.311481637390307,-0.848045003637591));
#123324=DIRECTION('ref_axis',(-0.892442058026276,-4.81426696315707E-15,
-0.451162025292273));
#123325=DIRECTION('center_axis',(-0.404512670528681,0.293895658256105,0.866022425483293));
#123326=DIRECTION('ref_axis',(0.906035197473496,4.3386129689956E-15,0.423202340422596));
#123327=DIRECTION('center_axis',(-0.428717658685243,0.311481638277357,0.848045021297512));
#123328=DIRECTION('ref_axis',(-0.683543400921194,0.501950189213663,-0.529919264233199));
#123329=DIRECTION('center_axis',(0.428717648856917,-0.311481604401037,-0.848045038708649));
#123330=DIRECTION('ref_axis',(-0.892442084777736,7.94801068170717E-15,-0.451161972375297));
#123331=DIRECTION('center_axis',(-0.404512675558581,0.293895674899355,0.866022417485766));
#123332=DIRECTION('ref_axis',(-0.69794602972004,0.512709800567571,-0.499999999999995));
#123333=DIRECTION('center_axis',(-0.70065917669006,0.509016097474051,0.499979330205054));
#123334=DIRECTION('ref_axis',(0.405058175799853,-0.29310044923218,0.866036951219513));
#123335=DIRECTION('center_axis',(0.587981418248444,0.808874435122379,0.));
#123336=DIRECTION('ref_axis',(-0.808874435122379,0.587981418248444,0.));
#123337=DIRECTION('center_axis',(0.809016994374943,-0.58778525229248,-1.13923270769252E-16));
#123338=DIRECTION('ref_axis',(0.58778525229248,0.809016994374943,4.71515639841956E-33));
#123339=DIRECTION('center_axis',(-0.809016994374912,0.587785252292522,0.));
#123340=DIRECTION('ref_axis',(-0.587785252292522,-0.809016994374912,0.));
#123341=DIRECTION('center_axis',(-2.54740177659162E-16,8.27701011433327E-17,
-1.));
#123342=DIRECTION('ref_axis',(-1.,-2.9359879547111E-33,2.25664243350207E-16));
#123343=DIRECTION('center_axis',(0.587589051772227,0.809159506053914,0.));
#123344=DIRECTION('ref_axis',(-0.809159506053914,0.587589051772227,0.));
#123345=DIRECTION('center_axis',(-0.428718069290599,0.31148190986391,-0.8480447139693));
#123346=DIRECTION('ref_axis',(-0.892441837073364,1.28712475779731E-15,0.451162462358205));
#123347=DIRECTION('center_axis',(-0.428717648856922,0.311481604401041,0.848045038708645));
#123348=DIRECTION('ref_axis',(0.892442084777733,-5.99017820001791E-15,0.451161972375302));
#123349=DIRECTION('center_axis',(-0.428718110499122,0.311481908632163,-0.848044693589275));
#123350=DIRECTION('ref_axis',(0.683410939224596,-0.502130522416956,-0.529919264233175));
#123351=DIRECTION('center_axis',(-0.428718122142699,0.311481948263265,-0.848044673146738));
#123352=DIRECTION('ref_axis',(-0.892441805934778,-4.37991823100416E-15,
0.451162523953256));
#123353=DIRECTION('center_axis',(0.428717658777127,-0.311481638420274,-0.848045021198569));
#123354=DIRECTION('ref_axis',(-0.688609525582563,0.494977266822919,-0.529919264233214));
#123355=DIRECTION('center_axis',(-0.428717694262775,0.311481637390324,0.848045003637574));
#123356=DIRECTION('ref_axis',(0.892442058026261,-6.4705373892766E-16,0.451162025292301));
#123357=DIRECTION('center_axis',(0.587994104813606,0.808865212939984,0.));
#123358=DIRECTION('ref_axis',(-0.808865212939984,0.587994104813606,0.));
#123359=DIRECTION('center_axis',(-0.809016994374931,0.587785252292496,0.));
#123360=DIRECTION('ref_axis',(-0.587785252292496,-0.809016994374931,0.));
#123361=DIRECTION('center_axis',(-2.54740177659162E-16,8.27701011433327E-17,
-1.));
#123362=DIRECTION('ref_axis',(-1.,-1.66692058590397E-33,2.40228573745067E-16));
#123363=DIRECTION('center_axis',(0.587576360591375,0.809168721883263,1.21071329521312E-14));
#123364=DIRECTION('ref_axis',(-0.809168721883263,0.587576360591375,1.5253418562395E-28));
#123365=DIRECTION('center_axis',(-0.809016994374943,0.58778525229248,1.13923270769252E-16));
#123366=DIRECTION('ref_axis',(-0.58778525229248,-0.809016994374943,-4.00133343489574E-31));
#123367=DIRECTION('center_axis',(-0.700605801485339,0.509057044367988,-0.500012436349751));
#123368=DIRECTION('ref_axis',(-0.405100113147179,0.293099122187947,0.866017784402143));
#123369=DIRECTION('center_axis',(0.428718122142675,-0.311481948263326,0.848044673146728));
#123370=DIRECTION('ref_axis',(0.892441805934786,-1.00097613656477E-15,-0.451162523953241));
#123371=DIRECTION('center_axis',(0.404512555982611,-0.293895562533576,0.866022511471548));
#123372=DIRECTION('ref_axis',(0.703251077796155,-0.505408667890181,-0.50000000000002));
#123373=DIRECTION('center_axis',(-0.404512560891349,0.293895578599941,-0.866022503726392));
#123374=DIRECTION('ref_axis',(-0.906035256115544,9.31541476348494E-16,0.423202214875631));
#123375=DIRECTION('center_axis',(0.428718110386438,-0.31148190845687,0.848044693710625));
#123376=DIRECTION('ref_axis',(0.688740099743675,-0.494795562227121,-0.529919264233166));
#123377=DIRECTION('center_axis',(0.428718069290549,-0.311481909863894,0.848044713969331));
#123378=DIRECTION('ref_axis',(0.892441837073392,-5.0994373414288E-15,-0.451162462358151));
#123379=DIRECTION('center_axis',(-0.809016994374931,0.587785252292496,0.));
#123380=DIRECTION('ref_axis',(-0.587785252292496,-0.809016994374931,0.));
#123381=DIRECTION('center_axis',(0.809016994374931,-0.587785252292496,0.));
#123382=DIRECTION('ref_axis',(0.587785252292496,0.809016994374931,0.));
#123383=DIRECTION('center_axis',(-0.809016994374943,0.58778525229248,1.13923270769252E-16));
#123384=DIRECTION('ref_axis',(-0.58778525229248,-0.809016994374943,-4.00133343489574E-31));
#123385=DIRECTION('center_axis',(-0.809016994374931,0.587785252292496,-1.08431827545695E-13));
#123386=DIRECTION('ref_axis',(-0.587785252292496,-0.809016994374931,-1.14793899448837E-30));
#123387=DIRECTION('center_axis',(-0.809016994374943,0.58778525229248,1.13923270769252E-16));
#123388=DIRECTION('ref_axis',(-0.58778525229248,-0.809016994374943,-4.00133343489574E-31));
#123389=DIRECTION('center_axis',(0.700618669263855,-0.509071851162735,-0.499979330205451));
#123390=DIRECTION('ref_axis',(-0.403924952201757,0.294660197705125,-0.86603695121928));
#123391=DIRECTION('center_axis',(-0.404512670528659,0.293895658256109,0.866022425483302));
#123392=DIRECTION('ref_axis',(0.906035197473505,-2.34802397371862E-15,0.423202340422577));
#123393=DIRECTION('center_axis',(-0.404512677789108,0.29389566353111,0.866022420301861));
#123394=DIRECTION('ref_axis',(0.587785252293696,0.809016994374059,8.74191355908437E-13));
#123395=DIRECTION('center_axis',(0.37157613913616,-0.334568658442753,0.866022508721616));
#123396=DIRECTION('ref_axis',(-0.669130606364157,-0.743144825472624,4.12618321919621E-12));
#123397=DIRECTION('center_axis',(0.643597063368368,-0.579456972966938,0.500012436348944));
#123398=DIRECTION('ref_axis',(0.37091925268088,-0.335308969592096,-0.86601778440269));
#123399=DIRECTION('center_axis',(-0.37157614556582,0.334568664232119,-0.866022503726309));
#123400=DIRECTION('ref_axis',(-0.918982183096524,2.56545002401075E-15,0.394299058014532));
#123401=DIRECTION('center_axis',(-0.743144825477379,0.669130606358875,0.));
#123402=DIRECTION('ref_axis',(-0.669130606358875,-0.743144825477379,0.));
#123403=DIRECTION('center_axis',(0.743144825477389,-0.669130606358864,-1.04647355694968E-16));
#123404=DIRECTION('ref_axis',(0.669130606358864,0.743144825477389,-1.94545925652658E-32));
#123405=DIRECTION('center_axis',(0.743144825477406,-0.669130606358845,4.06031740096479E-14));
#123406=DIRECTION('ref_axis',(0.669130606358845,0.743144825477406,-5.14555379104688E-31));
#123407=DIRECTION('center_axis',(0.743144825477389,-0.669130606358864,-1.04647355694968E-16));
#123408=DIRECTION('ref_axis',(0.669130606358864,0.743144825477389,-1.94545925652658E-32));
#123409=DIRECTION('center_axis',(-0.743144825477382,0.669130606358872,0.));
#123410=DIRECTION('ref_axis',(-0.669130606358872,-0.743144825477382,0.));
#123411=DIRECTION('center_axis',(0.393810436983645,-0.354588510146761,-0.848045003637573));
#123412=DIRECTION('ref_axis',(-0.90697822335776,9.40871057169973E-16,-0.421177518814575));
#123413=DIRECTION('center_axis',(-0.371576246276111,0.334568754912036,0.866022425483293));
#123414=DIRECTION('ref_axis',(0.918982131463648,2.13361091916559E-15,0.394299178353862));
#123415=DIRECTION('center_axis',(-0.393810401510386,0.354588507307772,0.848045021297498));
#123416=DIRECTION('ref_axis',(-0.627330796731871,0.570650194835957,-0.529919264233185));
#123417=DIRECTION('center_axis',(0.393810395274833,-0.354588472591978,-0.848045038708657));
#123418=DIRECTION('ref_axis',(-0.906978247051303,-9.32548843552878E-15,
-0.421177467792076));
#123419=DIRECTION('center_axis',(-0.37157624953287,0.334568771996355,0.866022417485793));
#123420=DIRECTION('ref_axis',(-0.640529840771603,0.582856348580999,-0.49999999999993));
#123421=DIRECTION('center_axis',(-0.64361422196112,0.579466481046826,0.499979330205351));
#123422=DIRECTION('ref_axis',(0.372201885186834,-0.333834922957544,0.866036951219345));
#123423=DIRECTION('center_axis',(0.669310796197597,0.742982542253409,0.));
#123424=DIRECTION('ref_axis',(-0.742982542253409,0.669310796197597,0.));
#123425=DIRECTION('center_axis',(0.743144825477389,-0.669130606358864,-1.04647355694968E-16));
#123426=DIRECTION('ref_axis',(0.669130606358864,0.743144825477389,-1.94545925652658E-32));
#123427=DIRECTION('center_axis',(-0.743144825477379,0.669130606358875,0.));
#123428=DIRECTION('ref_axis',(-0.669130606358875,-0.743144825477379,0.));
#123429=DIRECTION('center_axis',(-2.45464262584879E-16,9.42249022928256E-17,
-1.));
#123430=DIRECTION('ref_axis',(-1.,-2.34879036376888E-33,2.25664243350207E-16));
#123431=DIRECTION('center_axis',(0.668950377172438,0.743307065001304,0.));
#123432=DIRECTION('ref_axis',(-0.743307065001304,0.668950377172438,0.));
#123433=DIRECTION('center_axis',(-0.39381078147567,0.354588820328836,-0.848044713969332));
#123434=DIRECTION('ref_axis',(-0.906978027661857,7.54218793329778E-15,0.421177940232638));
#123435=DIRECTION('center_axis',(-0.393810395274846,0.35458847259199,0.848045038708646));
#123436=DIRECTION('ref_axis',(0.906978247051292,-8.75481591077838E-15,0.421177467792099));
#123437=DIRECTION('center_axis',(-0.39381082258445,0.354588823414425,-0.848044693589278));
#123438=DIRECTION('ref_axis',(0.627180210724977,-0.570815694133858,-0.529919264233199));
#123439=DIRECTION('center_axis',(-0.393810830024562,0.354588864042303,-0.848044673146736));
#123440=DIRECTION('ref_axis',(-0.906978000082633,-7.8483346287888E-15,0.421177999622614));
#123441=DIRECTION('center_axis',(0.393810401583025,-0.35458850746372,-0.848045021198561));
#123442=DIRECTION('ref_axis',(-0.633098037506084,0.56424502505606,-0.529919264233177));
#123443=DIRECTION('center_axis',(-0.393810436983627,0.354588510146745,0.848045003637588));
#123444=DIRECTION('ref_axis',(0.90697822335777,-1.33133695181472E-15,0.421177518814553));
#123445=DIRECTION('center_axis',(0.669322449283885,0.742972044483923,4.02398997762812E-15));
#123446=DIRECTION('ref_axis',(-0.742972044483923,0.669322449283885,8.69613941656436E-29));
#123447=DIRECTION('center_axis',(-0.743144825477406,0.669130606358845,0.));
#123448=DIRECTION('ref_axis',(-0.669130606358845,-0.743144825477406,0.));
#123449=DIRECTION('center_axis',(-2.45464262584879E-16,9.42249022928256E-17,
-1.));
#123450=DIRECTION('ref_axis',(-1.,-1.04182536618998E-33,2.40228573745067E-16));
#123451=DIRECTION('center_axis',(0.668938718831625,0.743317556935059,0.));
#123452=DIRECTION('ref_axis',(-0.743317556935059,0.668938718831625,0.));
#123453=DIRECTION('center_axis',(-0.743144825477389,0.669130606358864,1.04647355694968E-16));
#123454=DIRECTION('ref_axis',(-0.669130606358865,-0.743144825477389,8.32249373466419E-31));
#123455=DIRECTION('center_axis',(-0.643556859037426,0.579501624401081,-0.500012436347728));
#123456=DIRECTION('ref_axis',(-0.37224373150931,0.333837986827737,0.866017784403316));
#123457=DIRECTION('center_axis',(0.393810830024499,-0.354588864042362,0.848044673146741));
#123458=DIRECTION('ref_axis',(0.906978000082659,3.44782577783986E-15,-0.421177999622559));
#123459=DIRECTION('center_axis',(0.371576142361039,-0.334568647743098,0.866022511471523));
#123460=DIRECTION('ref_axis',(0.646569003432252,-0.576149740779758,-0.500000000000042));
#123461=DIRECTION('center_axis',(-0.371576145565792,0.33456866423203,-0.866022503726355));
#123462=DIRECTION('ref_axis',(-0.918982183096543,1.46372471911345E-15,0.394299058014488));
#123463=DIRECTION('center_axis',(0.393810822490023,-0.354588823229131,0.848044693710604));
#123464=DIRECTION('ref_axis',(0.633246889648164,-0.564077964598377,-0.529919264233221));
#123465=DIRECTION('center_axis',(0.393810781475714,-0.354588820328813,0.848044713969321));
#123466=DIRECTION('ref_axis',(0.906978027661839,8.40177352928018E-15,-0.421177940232677));
#123467=DIRECTION('center_axis',(-0.743144825477406,0.669130606358845,4.06031740096479E-14));
#123468=DIRECTION('ref_axis',(-0.669130606358845,-0.743144825477406,-5.14555379104688E-31));
#123469=DIRECTION('center_axis',(0.743144825477379,-0.669130606358875,0.));
#123470=DIRECTION('ref_axis',(0.669130606358875,0.743144825477379,0.));
#123471=DIRECTION('center_axis',(-0.743144825477389,0.669130606358864,1.04647355694968E-16));
#123472=DIRECTION('ref_axis',(-0.669130606358865,-0.743144825477389,8.32249373466419E-31));
#123473=DIRECTION('center_axis',(-0.743144825477406,0.669130606358845,4.06031740096457E-14));
#123474=DIRECTION('ref_axis',(-0.669130606358845,-0.743144825477406,2.80523855531594E-30));
#123475=DIRECTION('center_axis',(-0.743144825477389,0.669130606358864,1.04647355694968E-16));
#123476=DIRECTION('ref_axis',(-0.669130606358865,-0.743144825477389,8.32249373466419E-31));
#123477=DIRECTION('center_axis',(0.643568108591973,-0.579517695131666,-0.499979330205392));
#123478=DIRECTION('ref_axis',(-0.370911831395904,0.335267672842607,-0.866036951219311));
#123479=DIRECTION('center_axis',(-0.37157624627613,0.334568754912026,0.866022425483288));
#123480=DIRECTION('ref_axis',(0.918982131463641,8.64235197177631E-15,0.394299178353879));
#123481=DIRECTION('center_axis',(-0.37157625294445,0.334568760916253,0.866022420302572));
#123482=DIRECTION('ref_axis',(0.669130606362073,0.743144825474499,2.48270345075888E-12));
#123483=DIRECTION('center_axis',(0.33456865844238,-0.371576139135717,0.866022508721951));
#123484=DIRECTION('ref_axis',(-0.743144825474233,-0.669130606362369,-2.72747704315771E-12));
#123485=DIRECTION('center_axis',(0.579501624401054,-0.643556859037126,0.500012436348146));
#123486=DIRECTION('ref_axis',(0.333837986837391,-0.372243731501189,-0.866017784403085));
#123487=DIRECTION('center_axis',(-0.3345686642321,0.371576145565839,-0.866022503726308));
#123488=DIRECTION('ref_axis',(3.52929994070592E-15,0.918982183096517,0.394299058014547));
#123489=DIRECTION('center_axis',(-0.669130606358875,0.743144825477379,0.));
#123490=DIRECTION('ref_axis',(-0.743144825477379,-0.669130606358875,0.));
#123491=DIRECTION('center_axis',(0.669130606358852,-0.7431448254774,-9.42249022928238E-17));
#123492=DIRECTION('ref_axis',(0.7431448254774,0.669130606358852,-9.95814315644137E-34));
#123493=DIRECTION('center_axis',(0.669130606358845,-0.743144825477406,-3.65592620896146E-14));
#123494=DIRECTION('ref_axis',(0.743144825477406,0.669130606358845,9.99649599890217E-31));
#123495=DIRECTION('center_axis',(0.669130606358852,-0.7431448254774,-9.42249022928238E-17));
#123496=DIRECTION('ref_axis',(0.7431448254774,0.669130606358852,-9.95814315644137E-34));
#123497=DIRECTION('center_axis',(-0.669130606358845,0.743144825477406,0.));
#123498=DIRECTION('ref_axis',(-0.743144825477406,-0.669130606358845,0.));
#123499=DIRECTION('center_axis',(0.354588510146745,-0.393810436983627,-0.848045003637588));
#123500=DIRECTION('ref_axis',(-1.32348946953629E-15,0.90697822335777,-0.421177518814553));
#123501=DIRECTION('center_axis',(-0.334568754912041,0.371576246276148,0.866022425483275));
#123502=DIRECTION('ref_axis',(6.8466508941702E-15,-0.91898213146363,0.394299178353905));
#123503=DIRECTION('center_axis',(-0.354588475158959,0.393810430457258,0.848045021297521));
#123504=DIRECTION('ref_axis',(-0.564245025055314,0.633098037506755,-0.529919264233169));
#123505=DIRECTION('center_axis',(0.354588472592002,-0.39381039527486,-0.848045038708635));
#123506=DIRECTION('ref_axis',(-2.66687128082441E-15,0.906978247051286,-0.421177467792113));
#123507=DIRECTION('center_axis',(-0.334568756370059,0.371576263602952,0.866022417485749));
#123508=DIRECTION('ref_axis',(-0.576095872880217,0.646617000434065,-0.500000000000033));
#123509=DIRECTION('center_axis',(-0.579517695131992,0.643568108591923,0.499979330205078));
#123510=DIRECTION('ref_axis',(0.335267672822139,-0.370911831413928,0.866036951219515));
#123511=DIRECTION('center_axis',(0.743307065001336,0.668950377172403,0.));
#123512=DIRECTION('ref_axis',(-0.668950377172402,0.743307065001336,0.));
#123513=DIRECTION('center_axis',(0.669130606358852,-0.7431448254774,-9.42249022928238E-17));
#123514=DIRECTION('ref_axis',(0.7431448254774,0.669130606358852,-9.95814315644137E-34));
#123515=DIRECTION('center_axis',(-0.669130606358872,0.743144825477382,0.));
#123516=DIRECTION('ref_axis',(-0.743144825477382,-0.669130606358872,0.));
#123517=DIRECTION('center_axis',(-2.35041809182734E-16,1.0464735569497E-16,
-1.));
#123518=DIRECTION('ref_axis',(-1.,-1.56586024251259E-33,2.25664243350207E-16));
#123519=DIRECTION('center_axis',(0.742982542253406,0.669310796197601,0.));
#123520=DIRECTION('ref_axis',(-0.669310796197601,0.742982542253406,0.));
#123521=DIRECTION('center_axis',(-0.35458882032884,0.393810781475744,-0.848044713969297));
#123522=DIRECTION('ref_axis',(-2.60913257636008E-15,0.906978027661821,0.421177940232716));
#123523=DIRECTION('center_axis',(-0.354588472592004,0.393810395274862,0.848045038708633));
#123524=DIRECTION('ref_axis',(1.64363307278047E-15,-0.906978247051285,0.421177467792116));
#123525=DIRECTION('center_axis',(-0.35458886088619,0.393810788844712,-0.848044693589282));
#123526=DIRECTION('ref_axis',(0.564077964590569,-0.633246889655141,-0.529919264233195));
#123527=DIRECTION('center_axis',(-0.354588864042363,0.393810830024498,-0.848044673146741));
#123528=DIRECTION('ref_axis',(3.00368387037336E-15,0.90697800008266,0.421177999622557));
#123529=DIRECTION('center_axis',(0.354588475222375,-0.393810430613248,-0.848045021198568));
#123530=DIRECTION('ref_axis',(-0.570650194825298,0.627330796741533,-0.529919264233225));
#123531=DIRECTION('center_axis',(-0.354588510146774,0.393810436983659,0.848045003637561));
#123532=DIRECTION('ref_axis',(-5.40566344552556E-15,-0.906978223357753,
0.42117751881459));
#123533=DIRECTION('center_axis',(0.743317556935089,0.668938718831591,-4.06383359288233E-15));
#123534=DIRECTION('ref_axis',(-0.668938718831591,0.743317556935089,4.57642320323792E-30));
#123535=DIRECTION('center_axis',(-0.669130606358845,0.743144825477406,0.));
#123536=DIRECTION('ref_axis',(-0.743144825477406,-0.669130606358845,0.));
#123537=DIRECTION('center_axis',(-2.35041809182734E-16,1.0464735569497E-16,
-1.));
#123538=DIRECTION('ref_axis',(-1.,0.,2.40228573745067E-16));
#123539=DIRECTION('center_axis',(0.742972044483923,0.669322449283885,-4.02398997762833E-15));
#123540=DIRECTION('ref_axis',(-0.669322449283885,0.742972044483923,8.70403636810736E-29));
#123541=DIRECTION('center_axis',(-0.669130606358852,0.7431448254774,9.42249022928238E-17));
#123542=DIRECTION('ref_axis',(-0.7431448254774,-0.669130606358852,-8.60592964647315E-31));
#123543=DIRECTION('center_axis',(-0.579456972966213,0.643597063368616,-0.500012436349466));
#123544=DIRECTION('ref_axis',(-0.335308969664714,0.370919252616137,0.866017784402304));
#123545=DIRECTION('center_axis',(0.354588864042318,-0.393810830024549,0.848044673146736));
#123546=DIRECTION('ref_axis',(-3.66609196403161E-15,-0.906978000082638,
-0.421177999622604));
#123547=DIRECTION('center_axis',(0.334568662771634,-0.371576128829216,0.866022511471552));
#123548=DIRECTION('ref_axis',(0.582802983770213,-0.640578396535943,-0.499999999999977));
#123549=DIRECTION('center_axis',(-0.334568664232029,0.371576145565791,-0.866022503726356));
#123550=DIRECTION('ref_axis',(4.84407888932722E-15,0.918982183096544,0.394299058014485));
#123551=DIRECTION('center_axis',(0.354588860819346,-0.393810788643603,0.848044693710622));
#123552=DIRECTION('ref_axis',(0.570815694137047,-0.627180210722105,-0.529919264233163));
#123553=DIRECTION('center_axis',(0.354588820328778,-0.393810781475744,0.848044713969322));
#123554=DIRECTION('ref_axis',(6.08911365345571E-15,-0.906978027661825,-0.421177940232708));
#123555=DIRECTION('center_axis',(-0.669130606358845,0.743144825477406,-4.06031740096479E-14));
#123556=DIRECTION('ref_axis',(-0.743144825477406,-0.669130606358845,-1.17388982313054E-30));
#123557=DIRECTION('center_axis',(0.669130606358872,-0.743144825477382,0.));
#123558=DIRECTION('ref_axis',(0.743144825477382,0.669130606358872,0.));
#123559=DIRECTION('center_axis',(-0.669130606358852,0.7431448254774,9.42249022928238E-17));
#123560=DIRECTION('ref_axis',(-0.7431448254774,-0.669130606358852,-8.60592964647315E-31));
#123561=DIRECTION('center_axis',(-0.669130606358845,0.743144825477406,-3.65592620896146E-14));
#123562=DIRECTION('ref_axis',(-0.743144825477406,-0.669130606358845,9.99649599890217E-31));
#123563=DIRECTION('center_axis',(-0.669130606358852,0.7431448254774,9.42249022928238E-17));
#123564=DIRECTION('ref_axis',(-0.7431448254774,-0.669130606358852,-8.60592964647315E-31));
#123565=DIRECTION('center_axis',(0.579466481046707,-0.643614221961464,-0.499979330205044));
#123566=DIRECTION('ref_axis',(-0.333834922946263,0.372201885196569,-0.86603695121951));
#123567=DIRECTION('center_axis',(-0.334568754912033,0.371576246276138,0.866022425483283));
#123568=DIRECTION('ref_axis',(4.15067265588782E-15,-0.918982131463635,0.394299178353892));
#123569=DIRECTION('center_axis',(-0.334568760918544,0.37157625294706,0.866022420300568));
#123570=DIRECTION('ref_axis',(0.74314482547537,0.669130606361107,-1.78335036602841E-12));
#123571=DIRECTION('center_axis',(0.293895573515143,-0.404512553892808,0.866022508720948));
#123572=DIRECTION('ref_axis',(-0.809016994373897,-0.587785252293919,-1.08399728638205E-12));
#123573=DIRECTION('center_axis',(0.509057044367757,-0.700605801485709,0.500012436349469));
#123574=DIRECTION('ref_axis',(0.293099122173842,-0.405100113157068,-0.866017784402292));
#123575=DIRECTION('center_axis',(-0.293895578600024,0.404512560891464,-0.86602250372631));
#123576=DIRECTION('ref_axis',(5.57115822586198E-15,0.906035256115484,0.423202214875761));
#123577=DIRECTION('center_axis',(-0.58778525229247,0.80901699437495,0.));
#123578=DIRECTION('ref_axis',(-0.80901699437495,-0.58778525229247,0.));
#123579=DIRECTION('center_axis',(0.587785252292466,-0.809016994374953,-8.27701011433307E-17));
#123580=DIRECTION('ref_axis',(0.809016994374953,0.587785252292466,-1.11448779222234E-32));
#123581=DIRECTION('center_axis',(0.58778525229247,-0.80901699437495,0.));
#123582=DIRECTION('ref_axis',(0.80901699437495,0.58778525229247,0.));
#123583=DIRECTION('center_axis',(0.587785252292466,-0.809016994374953,-8.27701011433307E-17));
#123584=DIRECTION('ref_axis',(0.809016994374953,0.587785252292466,3.81297860563151E-33));
#123585=DIRECTION('center_axis',(-0.58778525229247,0.80901699437495,0.));
#123586=DIRECTION('ref_axis',(-0.80901699437495,-0.58778525229247,0.));
#123587=DIRECTION('center_axis',(0.311481637390299,-0.428717694262769,-0.848045003637586));
#123588=DIRECTION('ref_axis',(-4.11382121094243E-15,0.892442058026266,-0.451162025292292));
#123589=DIRECTION('center_axis',(-0.293895658256123,0.404512670528733,0.866022425483262));
#123590=DIRECTION('ref_axis',(-8.25691251523047E-15,-0.90603519747347,0.423202340422653));
#123591=DIRECTION('center_axis',(-0.311481603280472,0.428717684111969,0.848045021297511));
#123592=DIRECTION('ref_axis',(-0.494977266816266,0.688609525587369,-0.529919264233183));
#123593=DIRECTION('center_axis',(0.311481604401019,-0.428717648856921,-0.848045038708653));
#123594=DIRECTION('ref_axis',(-7.59295483192656E-15,0.892442084777736,-0.451161972375298));
#123595=DIRECTION('center_axis',(-0.293895657887586,0.404512687918341,0.866022417485773));
#123596=DIRECTION('ref_axis',(-0.505350078017002,0.703293181147248,-0.499999999999994));
#123597=DIRECTION('center_axis',(-0.509071851162815,0.700618669263933,0.49997933020526));
#123598=DIRECTION('ref_axis',(0.294660197713809,-0.403924952195204,0.866036951219381));
#123599=DIRECTION('center_axis',(0.809159506053914,0.587589051772227,0.));
#123600=DIRECTION('ref_axis',(-0.587589051772227,0.809159506053914,0.));
#123601=DIRECTION('center_axis',(0.587785252292466,-0.809016994374953,-8.27701011433307E-17));
#123602=DIRECTION('ref_axis',(0.809016994374953,0.587785252292466,-1.11448779222234E-32));
#123603=DIRECTION('center_axis',(-0.58778525229247,0.80901699437495,0.));
#123604=DIRECTION('ref_axis',(-0.80901699437495,-0.58778525229247,0.));
#123605=DIRECTION('center_axis',(-2.23587008033241E-16,1.13923270769253E-16,
-1.));
#123606=DIRECTION('ref_axis',(-1.,-3.91465060628147E-34,2.25664243350207E-16));
#123607=DIRECTION('center_axis',(0.808874435122379,0.587981418248444,0.));
#123608=DIRECTION('ref_axis',(-0.587981418248444,0.808874435122379,0.));
#123609=DIRECTION('center_axis',(-0.311481909863932,0.428718069290522,-0.848044713969331));
#123610=DIRECTION('ref_axis',(9.11251128025232E-15,0.892441837073405,0.451162462358124));
#123611=DIRECTION('center_axis',(-0.311481604401018,0.428717648856998,0.848045038708615));
#123612=DIRECTION('ref_axis',(2.45085461175841E-15,-0.892442084777695,0.451161972375377));
#123613=DIRECTION('center_axis',(-0.311481949435979,0.428718080853434,-0.848044693589265));
#123614=DIRECTION('ref_axis',(0.494795562220743,-0.688740099748264,-0.529919264233157));
#123615=DIRECTION('center_axis',(-0.311481948263276,0.428718122142686,-0.848044673146741));
#123616=DIRECTION('ref_axis',(2.81035723410834E-16,0.892441805934784,0.451162523953244));
#123617=DIRECTION('center_axis',(0.311481603324408,-0.428717684275746,-0.848045021198579));
#123618=DIRECTION('ref_axis',(-0.501950189202811,0.683543400929142,-0.529919264233227));
#123619=DIRECTION('center_axis',(-0.311481637390294,0.428717694262762,0.848045003637591));
#123620=DIRECTION('ref_axis',(6.8200989747602E-15,-0.89244205802627,0.451162025292285));
#123621=DIRECTION('center_axis',(0.809168721883286,0.587576360591345,-1.21071329521341E-14));
#123622=DIRECTION('ref_axis',(-0.587576360591345,0.809168721883286,-3.03871162902842E-28));
#123623=DIRECTION('center_axis',(-0.58778525229247,0.80901699437495,0.));
#123624=DIRECTION('ref_axis',(-0.80901699437495,-0.58778525229247,0.));
#123625=DIRECTION('center_axis',(-2.23587008033241E-16,1.13923270769253E-16,
-1.));
#123626=DIRECTION('ref_axis',(-1.,1.25019043942798E-33,2.40228573745067E-16));
#123627=DIRECTION('center_axis',(0.808865212939984,0.587994104813606,0.));
#123628=DIRECTION('ref_axis',(-0.587994104813606,0.808865212939984,0.));
#123629=DIRECTION('center_axis',(-0.587785252292466,0.809016994374953,8.27701011433307E-17));
#123630=DIRECTION('ref_axis',(-0.809016994374953,-0.587785252292466,-1.27906067821219E-31));
#123631=DIRECTION('center_axis',(-0.509008435042523,0.70064111822839,-0.500012436348571));
#123632=DIRECTION('ref_axis',(-0.294700492564884,0.403936649463788,0.866017784402828));
#123633=DIRECTION('center_axis',(0.31148194826325,-0.428718122142728,0.848044673146729));
#123634=DIRECTION('ref_axis',(7.04633136982833E-16,-0.892441805934763,-0.451162523953285));
#123635=DIRECTION('center_axis',(0.293895578900055,-0.40451254409162,0.866022511471571));
#123636=DIRECTION('ref_axis',(0.512651652657614,-0.697988741332897,-0.499999999999935));
#123637=DIRECTION('center_axis',(-0.293895578599974,0.404512560891423,-0.866022503726346));
#123638=DIRECTION('ref_axis',(3.81388142168972E-15,0.906035256115507,0.423202214875711));
#123639=DIRECTION('center_axis',(0.311481949380144,-0.428718080653948,0.848044693710621));
#123640=DIRECTION('ref_axis',(0.502130522403619,-0.683410939234349,-0.529919264233236));
#123641=DIRECTION('center_axis',(0.311481909863867,-0.428718069290581,0.848044713969325));
#123642=DIRECTION('ref_axis',(-4.71143346943765E-15,-0.892441837073378,
-0.451162462358177));
#123643=DIRECTION('center_axis',(-0.58778525229247,0.80901699437495,0.));
#123644=DIRECTION('ref_axis',(-0.80901699437495,-0.58778525229247,0.));
#123645=DIRECTION('center_axis',(0.587785252292496,-0.809016994374931,0.));
#123646=DIRECTION('ref_axis',(0.809016994374931,0.587785252292496,0.));
#123647=DIRECTION('center_axis',(-0.587785252292466,0.809016994374953,8.27701011433307E-17));
#123648=DIRECTION('ref_axis',(-0.809016994374953,-0.587785252292466,-1.27906067821219E-31));
#123649=DIRECTION('center_axis',(-0.58778525229247,0.80901699437495,1.20874298148573E-14));
#123650=DIRECTION('ref_axis',(-0.80901699437495,-0.58778525229247,-1.84071433653408E-31));
#123651=DIRECTION('center_axis',(-0.587785252292466,0.809016994374953,8.27701011433307E-17));
#123652=DIRECTION('ref_axis',(-0.809016994374953,-0.587785252292466,-1.27906067821219E-31));
#123653=DIRECTION('center_axis',(0.509016097474312,-0.700659176689658,-0.499979330205352));
#123654=DIRECTION('ref_axis',(-0.293100449226779,0.405058175804142,-0.866036951219335));
#123655=DIRECTION('center_axis',(-0.293895658256093,0.404512670528665,0.866022425483304));
#123656=DIRECTION('ref_axis',(1.1317083799287E-15,-0.906035197473503,0.42320234042258));
#123657=DIRECTION('center_axis',(-0.293895663531789,0.404512677790057,0.866022420301188));
#123658=DIRECTION('ref_axis',(0.809016994371241,0.587785252297575,-3.67160369476059E-12));
#123659=DIRECTION('center_axis',(0.250002507181632,-0.433017044458199,0.866022508721098));
#123660=DIRECTION('ref_axis',(-0.866025403784408,-0.500000000000054,-3.49676543996346E-14));
#123661=DIRECTION('center_axis',(0.433035128829457,-0.749978760163043,0.500012436349297));
#123662=DIRECTION('ref_axis',(0.249149002268627,-0.433518133146968,-0.866017784402443));
#123663=DIRECTION('center_axis',(-0.25000251150716,0.433017051950293,-0.866022503726312));
#123664=DIRECTION('ref_axis',(3.51864076615538E-15,0.894424794863778,0.447218387740138));
#123665=DIRECTION('center_axis',(-0.500000000000022,0.866025403784426,0.));
#123666=DIRECTION('ref_axis',(-0.866025403784426,-0.500000000000022,0.));
#123667=DIRECTION('center_axis',(0.499999999999992,-0.866025403784443,-7.04084534449541E-17));
#123668=DIRECTION('ref_axis',(0.866025403784443,0.499999999999992,-1.7712134304101E-32));
#123669=DIRECTION('center_axis',(0.50000000000001,-0.866025403784433,1.36592399683214E-14));
#123670=DIRECTION('ref_axis',(0.866025403784433,0.50000000000001,3.78074180857848E-32));
#123671=DIRECTION('center_axis',(0.499999999999992,-0.866025403784443,-7.04084534449541E-17));
#123672=DIRECTION('ref_axis',(0.866025403784443,0.499999999999992,-1.7712134304101E-32));
#123673=DIRECTION('center_axis',(-0.50000000000001,0.866025403784433,0.));
#123674=DIRECTION('ref_axis',(-0.866025403784433,-0.50000000000001,0.));
#123675=DIRECTION('center_axis',(0.264962106632875,-0.45892783076861,-0.848045003637594));
#123676=DIRECTION('ref_axis',(-1.43964512713556E-15,0.879478602053341,-0.475938429348064));
#123677=DIRECTION('center_axis',(-0.25000257926675,0.433017169313245,0.866022425483265));
#123678=DIRECTION('ref_axis',(-1.3082911094407E-15,-0.8944247302164,0.44721851703314));
#123679=DIRECTION('center_axis',(-0.264962073769681,0.458927817108741,0.848045021297499));
#123680=DIRECTION('ref_axis',(-0.42028643404606,0.736576463614905,-0.529919264233154));
#123681=DIRECTION('center_axis',(0.264962078570529,-0.458927782163201,-0.848045038708647));
#123682=DIRECTION('ref_axis',(-1.89361858943742E-15,0.879478631391252,-0.475938375135028));
#123683=DIRECTION('center_axis',(-0.250002577084016,0.433017186568188,0.866022417485784));
#123684=DIRECTION('ref_axis',(-0.429067561962739,0.752263934581071,-0.499999999999957));
#123685=DIRECTION('center_axis',(-0.433048509462457,0.749993105181608,0.499979330205154));
#123686=DIRECTION('ref_axis',(0.250824363778504,-0.432512586704271,0.866036951219455));
#123687=DIRECTION('center_axis',(0.866146626230631,0.499789977759954,0.));
#123688=DIRECTION('ref_axis',(-0.499789977759954,0.866146626230631,0.));
#123689=DIRECTION('center_axis',(0.499999999999992,-0.866025403784443,-7.04084534449541E-17));
#123690=DIRECTION('ref_axis',(0.866025403784443,0.499999999999992,-1.7712134304101E-32));
#123691=DIRECTION('center_axis',(-0.499999999999998,0.86602540378444,0.));
#123692=DIRECTION('ref_axis',(-0.86602540378444,-0.499999999999998,0.));
#123693=DIRECTION('center_axis',(-2.11225360334865E-16,1.21951018649011E-16,
-1.));
#123694=DIRECTION('ref_axis',(-1.,1.17439518188444E-33,2.25664243350207E-16));
#123695=DIRECTION('center_axis',(0.865904130412297,0.500209992837931,0.));
#123696=DIRECTION('ref_axis',(-0.500209992837931,0.865904130412297,0.));
#123697=DIRECTION('center_axis',(-0.264962338412774,0.458928232223215,-0.848044713969322));
#123698=DIRECTION('ref_axis',(6.42968295905551E-16,0.87947835973774,0.475938877118706));
#123699=DIRECTION('center_axis',(-0.264962078570521,0.458927782163201,0.848045038708649));
#123700=DIRECTION('ref_axis',(2.043795734415E-15,-0.879478631391252,0.475938375135027));
#123701=DIRECTION('center_axis',(-0.264962376552941,0.45892824786285,-0.84804469358929));
#123702=DIRECTION('ref_axis',(0.420092076162084,-0.736687329156922,-0.529919264233213));
#123703=DIRECTION('center_axis',(-0.264962371077221,0.458928288799652,-0.848044673146739));
#123704=DIRECTION('ref_axis',(-5.61404975480703E-15,0.87947832558851,0.475938940222411));
#123705=DIRECTION('center_axis',(0.264962073787568,-0.458927817281253,-0.848045021198554));
#123706=DIRECTION('ref_axis',(-0.427750712267922,0.732266960574363,-0.529919264233213));
#123707=DIRECTION('center_axis',(-0.264962106632886,0.458927830768643,0.848045003637573));
#123708=DIRECTION('ref_axis',(3.30353726242757E-15,-0.879478602053321,0.4759384293481));
#123709=DIRECTION('center_axis',(0.86615446498511,0.499776392786171,0.));
#123710=DIRECTION('ref_axis',(-0.499776392786171,0.86615446498511,0.));
#123711=DIRECTION('center_axis',(-0.50000000000001,0.866025403784433,0.));
#123712=DIRECTION('ref_axis',(-0.866025403784433,-0.50000000000001,0.));
#123713=DIRECTION('center_axis',(-2.11225360334865E-16,1.21951018649011E-16,
-1.));
#123714=DIRECTION('ref_axis',(-1.,2.81292848871296E-33,2.40228573745067E-16));
#123715=DIRECTION('center_axis',(0.865896284857143,0.500223573885315,-2.73306953340429E-14));
#123716=DIRECTION('ref_axis',(-0.500223573885315,0.865896284857143,-4.47025834271801E-28));
#123717=DIRECTION('center_axis',(-0.499999999999992,0.866025403784443,7.04084534449541E-17));
#123718=DIRECTION('ref_axis',(-0.866025403784443,-0.499999999999992,-6.94743527014557E-31));
#123719=DIRECTION('center_axis',(-0.432983094185233,0.750008802378944,-0.500012436349222));
#123720=DIRECTION('ref_axis',(-0.250863215139369,0.43252843188453,0.866017784402519));
#123721=DIRECTION('center_axis',(0.264962371077185,-0.458928288799684,0.848044673146733));
#123722=DIRECTION('ref_axis',(-2.53116482579111E-15,-0.879478325588496,
-0.475938940222437));
#123723=DIRECTION('center_axis',(0.250002513560361,-0.433017035274593,0.866022511471557));
#123724=DIRECTION('ref_axis',(0.436883602752815,-0.747751775421316,-0.499999999999991));
#123725=DIRECTION('center_axis',(-0.250002511507164,0.43301705195022,-0.866022503726347));
#123726=DIRECTION('ref_axis',(-4.94285822981357E-15,0.894424794863815,0.447218387740065));
#123727=DIRECTION('center_axis',(0.264962376523978,-0.458928247655394,0.848044693710606));
#123728=DIRECTION('ref_axis',(0.427943903610924,-0.732154074465734,-0.529919264233212));
#123729=DIRECTION('center_axis',(0.264962338412787,-0.458928232223194,0.848044713969329));
#123730=DIRECTION('ref_axis',(5.019182273909E-15,-0.87947835973775,-0.475938877118687));
#123731=DIRECTION('center_axis',(-0.50000000000001,0.866025403784433,6.09762352041363E-14));
#123732=DIRECTION('ref_axis',(-0.866025403784433,-0.50000000000001,2.00105264687255E-32));
#123733=DIRECTION('center_axis',(0.499999999999998,-0.86602540378444,0.));
#123734=DIRECTION('ref_axis',(0.86602540378444,0.499999999999998,0.));
#123735=DIRECTION('center_axis',(-0.499999999999992,0.866025403784443,7.04084534449541E-17));
#123736=DIRECTION('ref_axis',(-0.866025403784443,-0.499999999999992,-6.94743527014557E-31));
#123737=DIRECTION('center_axis',(-0.50000000000001,0.866025403784433,-2.73184799366427E-14));
#123738=DIRECTION('ref_axis',(-0.866025403784433,-0.50000000000001,-7.56148361715697E-32));
#123739=DIRECTION('center_axis',(-0.499999999999992,0.866025403784443,7.04084534449541E-17));
#123740=DIRECTION('ref_axis',(-0.866025403784443,-0.499999999999992,-6.94743527014557E-31));
#123741=DIRECTION('center_axis',(0.432988827019321,-0.750027562856135,-0.499979330205279));
#123742=DIRECTION('ref_axis',(-0.249154705643646,0.433476564278025,-0.866036951219373));
#123743=DIRECTION('center_axis',(-0.250002579266693,0.433017169313166,0.866022425483321));
#123744=DIRECTION('ref_axis',(-6.80109926771202E-15,-0.894424730216445,
0.447218517033049));
#123745=DIRECTION('center_axis',(-0.250002583755051,0.433017177087239,0.866022420300536));
#123746=DIRECTION('ref_axis',(0.866025403785887,0.499999999997491,1.67844740332471E-12));
#123747=DIRECTION('center_axis',(0.203370361064481,-0.456777309673029,0.866022508719244));
#123748=DIRECTION('ref_axis',(-0.913545457641425,-0.406736643078441,-1.67844741116904E-12));
#123749=DIRECTION('center_axis',(0.352268789800274,-0.791134794601849,0.500012436348278));
#123750=DIRECTION('ref_axis',(0.202469153659259,-0.457186437806557,-0.866017784402985));
#123751=DIRECTION('center_axis',(-0.203370364581913,0.456777317573275,-0.866022503726308));
#123752=DIRECTION('ref_axis',(-5.36134519175288E-15,0.884507036382097,0.466526850878446));
#123753=DIRECTION('center_axis',(-0.406736643075807,0.913545457642598,0.));
#123754=DIRECTION('ref_axis',(-0.913545457642598,-0.406736643075807,0.));
#123755=DIRECTION('center_axis',(0.406736643075792,-0.913545457642605,-5.72753959967185E-17));
#123756=DIRECTION('ref_axis',(0.913545457642605,0.406736643075792,-7.24473849677094E-34));
#123757=DIRECTION('center_axis',(0.406736643075807,-0.913545457642598,0.));
#123758=DIRECTION('ref_axis',(0.913545457642598,0.406736643075807,0.));
#123759=DIRECTION('center_axis',(0.406736643075792,-0.913545457642605,-5.72753959967185E-17));
#123760=DIRECTION('ref_axis',(0.913545457642605,0.406736643075792,-7.24473849677094E-34));
#123761=DIRECTION('center_axis',(-0.406736643075751,0.913545457642623,0.));
#123762=DIRECTION('ref_axis',(-0.913545457642623,-0.406736643075751,0.));
#123763=DIRECTION('center_axis',(0.215539595588322,-0.484109857923806,-0.848045003637552));
#123764=DIRECTION('ref_axis',(-1.22051060460069E-15,0.868458021515973,-0.495762710240052));
#123765=DIRECTION('center_axis',(-0.20337041970245,0.456777441376077,0.866022425483297));
#123766=DIRECTION('ref_axis',(2.19291865361494E-15,-0.884506966812057,0.466526982779061));
#123767=DIRECTION('center_axis',(-0.215539564334464,0.484109840902905,0.848045021297498));
#123768=DIRECTION('ref_axis',(-0.340990855184624,0.776473315752058,-0.529919264233207));
#123769=DIRECTION('center_axis',(0.215539572760323,-0.484109806651279,-0.848045038708652));
#123770=DIRECTION('ref_axis',(-1.14521404331846E-15,0.868458052949962,-0.495762655175196));
#123771=DIRECTION('center_axis',(-0.203370415731982,0.456777458306689,0.866022417485761));
#123772=DIRECTION('ref_axis',(-0.348084091918818,0.792992726923176,-0.499999999999997));
#123773=DIRECTION('center_axis',(-0.352280597671314,0.791150459692796,0.499979330204979));
#123774=DIRECTION('ref_axis',(0.204240445642938,-0.456361522792971,0.866036951219551));
#123775=DIRECTION('center_axis',(0.913644062717554,0.406515100163527,-2.49593669965817E-14));
#123776=DIRECTION('ref_axis',(-0.406515100163527,0.913644062717554,2.93346074380205E-28));
#123777=DIRECTION('center_axis',(0.406736643075792,-0.913545457642605,-5.72753959967185E-17));
#123778=DIRECTION('ref_axis',(0.913545457642605,0.406736643075792,-7.24473849677094E-34));
#123779=DIRECTION('center_axis',(-0.406736643075807,0.913545457642598,0.));
#123780=DIRECTION('ref_axis',(-0.913545457642598,-0.406736643075807,0.));
#123781=DIRECTION('center_axis',(-1.98092302886629E-16,1.28642645648559E-16,
-1.));
#123782=DIRECTION('ref_axis',(-1.,2.74025542439703E-33,2.25664243350207E-16));
#123783=DIRECTION('center_axis',(0.913446798847323,0.406958162070229,0.));
#123784=DIRECTION('ref_axis',(-0.406958162070229,0.913446798847323,0.));
#123785=DIRECTION('center_axis',(-0.215539784135063,0.484110281406767,-0.8480447139693));
#123786=DIRECTION('ref_axis',(-1.11523192825129E-16,0.868457761888259,0.495763165045606));
#123787=DIRECTION('center_axis',(-0.215539572760323,0.484109806651281,0.848045038708651));
#123788=DIRECTION('ref_axis',(6.78208419898497E-16,-0.868458052949962,0.495762655175198));
#123789=DIRECTION('center_axis',(-0.215539820430813,0.484110300947715,-0.848044693589297));
#123790=DIRECTION('ref_axis',(0.340785973389205,-0.776563258038715,-0.529919264233212));
#123791=DIRECTION('center_axis',(-0.215539810706713,0.484110341087608,-0.848044673146736));
#123792=DIRECTION('ref_axis',(-4.23381048949575E-15,0.86845772529927,0.495763229140704));
#123793=DIRECTION('center_axis',(0.215539564338691,-0.484109841074344,-0.848045021198557));
#123794=DIRECTION('ref_axis',(-0.348864709029164,0.772967650156545,-0.529919264233209));
#123795=DIRECTION('center_axis',(-0.215539595588306,0.48410985792377,0.848045003637576));
#123796=DIRECTION('ref_axis',(5.65310087418454E-16,-0.868458021515995,0.495762710240013));
#123797=DIRECTION('center_axis',(0.913650438514074,0.406500770236713,0.));
#123798=DIRECTION('ref_axis',(-0.406500770236713,0.913650438514073,0.));
#123799=DIRECTION('center_axis',(-0.406736643075807,0.913545457642598,3.88019196882762E-14));
#123800=DIRECTION('ref_axis',(-0.913545457642598,-0.406736643075807,-7.82081982317031E-31));
#123801=DIRECTION('center_axis',(-1.98092302886629E-16,1.28642645648559E-16,
-1.));
#123802=DIRECTION('ref_axis',(-1.,4.68821414785493E-33,2.40228573745067E-16));
#123803=DIRECTION('center_axis',(0.913440415876957,0.406972488803028,-2.49538036744541E-14));
#123804=DIRECTION('ref_axis',(-0.406972488803028,0.913440415876957,1.34873736753699E-28));
#123805=DIRECTION('center_axis',(-0.406736643075792,0.913545457642605,5.72753959967185E-17));
#123806=DIRECTION('ref_axis',(-0.913545457642605,-0.406736643075792,-5.10634159526644E-31));
#123807=DIRECTION('center_axis',(-0.352213899942141,0.7911592331408,-0.500012436348947));
#123808=DIRECTION('ref_axis',(-0.204277427990782,0.456381342203981,0.866017784402586));
#123809=DIRECTION('center_axis',(0.215539810706706,-0.484110341087606,0.848044673146739));
#123810=DIRECTION('ref_axis',(4.86428769523775E-15,-0.868457725299271,-0.495763229140701));
#123811=DIRECTION('center_axis',(0.203370368362508,-0.456777301205554,0.866022511471537));
#123812=DIRECTION('ref_axis',(0.35632896466816,-0.789322284582468,-0.500000000000031));
#123813=DIRECTION('center_axis',(-0.203370364581893,0.456777317573231,-0.866022503726336));
#123814=DIRECTION('ref_axis',(-1.22569712450493E-15,0.884507036382122,0.466526850878399));
#123815=DIRECTION('center_axis',(0.215539820427113,-0.484110300736857,0.848044693710607));
#123816=DIRECTION('ref_axis',(0.349068641869984,-0.772875576440095,-0.529919264233181));
#123817=DIRECTION('center_axis',(0.215539784134997,-0.48411028140675,0.848044713969326));
#123818=DIRECTION('ref_axis',(-3.99144860726419E-15,-0.868457761888273,
-0.495763165045581));
#123819=DIRECTION('center_axis',(-0.406736643075807,0.913545457642598,1.11114268233636E-14));
#123820=DIRECTION('ref_axis',(-0.913545457642598,-0.406736643075807,-1.88066567154315E-32));
#123821=DIRECTION('center_axis',(0.406736643075751,-0.913545457642623,0.));
#123822=DIRECTION('ref_axis',(0.913545457642623,0.406736643075751,0.));
#123823=DIRECTION('center_axis',(-0.406736643075792,0.913545457642605,5.72753959967185E-17));
#123824=DIRECTION('ref_axis',(-0.913545457642605,-0.406736643075792,-5.10634159526644E-31));
#123825=DIRECTION('center_axis',(-0.406736643075807,0.913545457642598,2.76904928649126E-14));
#123826=DIRECTION('ref_axis',(-0.913545457642598,-0.406736643075807,1.39870556442785E-30));
#123827=DIRECTION('center_axis',(-0.406736643075792,0.913545457642605,5.72753959967185E-17));
#123828=DIRECTION('ref_axis',(-0.913545457642605,-0.406736643075792,-5.10634159526644E-31));
#123829=DIRECTION('center_axis',(0.352217640366456,-0.791178490090896,-0.499979330204935));
#123830=DIRECTION('ref_axis',(-0.202479170974534,0.457145692798004,-0.866036951219576));
#123831=DIRECTION('center_axis',(-0.203370419702469,0.45677744137607,0.866022425483297));
#123832=DIRECTION('ref_axis',(-6.1956980622853E-15,-0.884506966812061,0.466526982779054));
#123833=DIRECTION('center_axis',(-0.203370423351418,0.456777449571772,0.866022420303639));
#123834=DIRECTION('ref_axis',(0.913545457643787,0.406736643073135,1.67844740332474E-12));
#123835=DIRECTION('center_axis',(0.154510046710178,-0.475533027088194,0.866022508722469));
#123836=DIRECTION('ref_axis',(-0.951056516294165,-0.309016994377989,-1.85328568317356E-12));
#123837=DIRECTION('center_axis',(0.267642920194485,-0.823622990674322,0.500012436347791));
#123838=DIRECTION('ref_axis',(0.153571010689768,-0.475845712151499,-0.866017784403274));
#123839=DIRECTION('center_axis',(-0.154510049384264,0.475533035318155,-0.866022503726303));
#123840=DIRECTION('ref_axis',(-4.8539766534288E-15,0.876548788012427,0.481313018974082));
#123841=DIRECTION('center_axis',(-0.309016994374914,0.951056516295165,0.));
#123842=DIRECTION('ref_axis',(-0.951056516295164,-0.309016994374914,0.));
#123843=DIRECTION('center_axis',(0.309016994374938,-0.951056516295157,-4.35148173242957E-17));
#123844=DIRECTION('ref_axis',(0.951056516295157,0.309016994374938,-2.85097203607405E-33));
#123845=DIRECTION('center_axis',(0.309016994374914,-0.951056516295164,-6.04047112789604E-14));
#123846=DIRECTION('ref_axis',(0.951056516295164,0.309016994374914,2.74316558509634E-30));
#123847=DIRECTION('center_axis',(0.309016994374938,-0.951056516295157,-4.35148173242957E-17));
#123848=DIRECTION('ref_axis',(0.951056516295157,0.309016994374938,-2.85097203607405E-33));
#123849=DIRECTION('center_axis',(-0.30901699437498,0.951056516295143,0.));
#123850=DIRECTION('ref_axis',(-0.951056516295143,-0.30901699437498,0.));
#123851=DIRECTION('center_axis',(0.163755587629875,-0.503987876168985,-0.848045003637584));
#123852=DIRECTION('ref_axis',(3.02936709568593E-15,0.859649462041489,-0.510884333691862));
#123853=DIRECTION('center_axis',(-0.154510091261946,0.475533164204408,0.866022425483295));
#123854=DIRECTION('ref_axis',(-2.02831240586475E-15,-0.876548714628839,
0.481313152617431));
#123855=DIRECTION('center_axis',(-0.163755558330189,0.50398785597322,0.848045021297505));
#123856=DIRECTION('ref_axis',(-0.25795930913709,0.807862963765557,-0.52991926423319));
#123857=DIRECTION('center_axis',(0.163755570286389,-0.503987822791223,-0.848045038708642));
#123858=DIRECTION('ref_axis',(-4.55251793567526E-15,0.859649495083692,-0.510884278092753));
#123859=DIRECTION('center_axis',(-0.154510085538992,0.475533180628678,0.866022417485775));
#123860=DIRECTION('ref_axis',(-0.263286939707607,0.825033325011428,-0.49999999999999));
#123861=DIRECTION('center_axis',(-0.267653025932399,0.823639804208775,0.49997933020492));
#123862=DIRECTION('ref_axis',(0.155418826433078,-0.475210466543448,0.86603695121959));
#123863=DIRECTION('center_axis',(0.951131423661017,0.308786358060986,0.));
#123864=DIRECTION('ref_axis',(-0.308786358060986,0.951131423661017,0.));
#123865=DIRECTION('center_axis',(0.309016994374938,-0.951056516295157,-4.35148173242957E-17));
#123866=DIRECTION('ref_axis',(0.951056516295157,0.309016994374938,-2.85097203607405E-33));
#123867=DIRECTION('center_axis',(-0.309016994374914,0.951056516295165,0.));
#123868=DIRECTION('ref_axis',(-0.951056516295164,-0.309016994374914,0.));
#123869=DIRECTION('center_axis',(-1.84331724214206E-16,1.33924836902178E-16,
-1.));
#123870=DIRECTION('ref_axis',(-1.,4.69758072753777E-33,2.25664243350207E-16));
#123871=DIRECTION('center_axis',(0.95098155300316,0.309247612517378,0.));
#123872=DIRECTION('ref_axis',(-0.309247612517378,0.95098155300316,0.));
#123873=DIRECTION('center_axis',(-0.163755730877748,0.503988317040607,-0.848044713969299));
#123874=DIRECTION('ref_axis',(5.60887131859091E-15,0.859649189130451,0.510884792910651));
#123875=DIRECTION('center_axis',(-0.163755570286382,0.503987822791203,0.848045038708655));
#123876=DIRECTION('ref_axis',(9.71142862414541E-16,-0.859649495083705,0.510884278092731));
#123877=DIRECTION('center_axis',(-0.163755764938156,0.503988340266509,-0.848044693589276));
#123878=DIRECTION('ref_axis',(0.257746148170087,-0.8079309973618,-0.529919264233195));
#123879=DIRECTION('center_axis',(-0.163755751065481,0.503988379172012,-0.848044673146732));
#123880=DIRECTION('ref_axis',(-4.45972261711213E-15,0.85964915066946,0.510884857627701));
#123881=DIRECTION('center_axis',(0.163755558314818,-0.503987856144707,-0.848045021198559));
#123882=DIRECTION('ref_axis',(-0.266156471020442,0.805199544416449,-0.52991926423323));
#123883=DIRECTION('center_axis',(-0.163755587629886,0.50398787616902,0.848045003637562));
#123884=DIRECTION('ref_axis',(-2.19355421648303E-15,-0.859649462041468,
0.510884333691899));
#123885=DIRECTION('center_axis',(0.951136266645031,0.308771440182787,-1.68703327872841E-14));
#123886=DIRECTION('ref_axis',(-0.308771440182787,0.951136266645031,1.33674482860247E-28));
#123887=DIRECTION('center_axis',(-0.309016994374914,0.951056516295165,0.));
#123888=DIRECTION('ref_axis',(-0.951056516295164,-0.309016994374914,0.));
#123889=DIRECTION('center_axis',(-1.84331724214206E-16,1.33924836902178E-16,
-1.));
#123890=DIRECTION('ref_axis',(-1.,6.6676823436159E-33,2.40228573745067E-16));
#123891=DIRECTION('center_axis',(0.950976702550726,0.309262527968953,-1.68971643309511E-14));
#123892=DIRECTION('ref_axis',(-0.309262527968953,0.950976702550726,2.53399383097093E-28));
#123893=DIRECTION('center_axis',(-0.309016994374938,0.951056516295157,4.35148173242957E-17));
#123894=DIRECTION('ref_axis',(-0.951056516295156,-0.309016994374938,1.19291088153759E-31));
#123895=DIRECTION('center_axis',(-0.267585776504812,0.823641557783688,-0.500012436349313));
#123896=DIRECTION('ref_axis',(-0.15545353440973,0.475234043117894,0.866017784402458));
#123897=DIRECTION('center_axis',(0.163755751065396,-0.503988379172023,0.848044673146743));
#123898=DIRECTION('ref_axis',(3.85968722528993E-15,-0.859649150669458,-0.510884857627704));
#123899=DIRECTION('center_axis',(0.154510054856149,-0.475533019434887,0.866022511471549));
#123900=DIRECTION('ref_axis',(0.271870311899548,-0.822244813609475,-0.499999999999963));
#123901=DIRECTION('center_axis',(-0.154510049384232,0.475533035318044,-0.86602250372637));
#123902=DIRECTION('ref_axis',(5.01558990523659E-15,0.876548788012491,0.481313018973966));
#123903=DIRECTION('center_axis',(0.163755764945469,-0.503988340060009,0.848044693710586));
#123904=DIRECTION('ref_axis',(0.266368911006386,-0.805129291880355,-0.52991926423325));
#123905=DIRECTION('center_axis',(0.163755730877703,-0.503988317040573,0.848044713969329));
#123906=DIRECTION('ref_axis',(1.7121350261526E-15,-0.859649189130473,-0.510884792910613));
#123907=DIRECTION('center_axis',(-0.309016994374914,0.951056516295164,8.44187456091302E-15));
#123908=DIRECTION('ref_axis',(-0.951056516295164,-0.309016994374914,-8.17628747588762E-32));
#123909=DIRECTION('center_axis',(0.309016994374914,-0.951056516295165,0.));
#123910=DIRECTION('ref_axis',(0.951056516295164,0.309016994374914,0.));
#123911=DIRECTION('center_axis',(-0.309016994374938,0.951056516295157,4.35148173242957E-17));
#123912=DIRECTION('ref_axis',(-0.951056516295156,-0.309016994374938,1.19291088153759E-31));
#123913=DIRECTION('center_axis',(-0.309016994374914,0.951056516295164,-8.44187456091302E-15));
#123914=DIRECTION('ref_axis',(-0.951056516295164,-0.309016994374914,8.17628747588762E-32));
#123915=DIRECTION('center_axis',(-0.309016994374938,0.951056516295157,4.35148173242957E-17));
#123916=DIRECTION('ref_axis',(-0.951056516295156,-0.309016994374938,1.19291088153759E-31));
#123917=DIRECTION('center_axis',(0.267587483540081,-0.823661100222712,-0.499979330205359));
#123918=DIRECTION('ref_axis',(-0.153585232144589,0.475806237443143,-0.866036951219342));
#123919=DIRECTION('center_axis',(-0.154510091261949,0.475533164204404,0.866022425483296));
#123920=DIRECTION('ref_axis',(-1.35777311912048E-15,-0.876548714628841,
0.481313152617427));
#123921=DIRECTION('center_axis',(-0.154510094035502,0.475533172740419,0.866022420301328));
#123922=DIRECTION('ref_axis',(0.951056516294199,0.309016994377886,-1.78335036603156E-12));
#123923=DIRECTION('center_axis',(0.103956887954197,-0.489078705157028,0.866022508719493));
#123924=DIRECTION('ref_axis',(-0.978147600733613,-0.207911690818664,-5.24514815992741E-13));
#123925=DIRECTION('center_axis',(0.180084698745668,-0.847087400906779,0.500012436348017));
#123926=DIRECTION('ref_axis',(0.102990311633872,-0.489291521290677,-0.866017784403192));
#123927=DIRECTION('center_axis',(-0.103956889752271,0.48907871361637,-0.866022503726313));
#123928=DIRECTION('ref_axis',(-1.92726867033915E-15,0.870740345484703,0.491743073916837));
#123929=DIRECTION('center_axis',(-0.207911690817757,0.978147600733806,0.));
#123930=DIRECTION('ref_axis',(-0.978147600733806,-0.207911690817757,0.));
#123931=DIRECTION('center_axis',(0.207911690817749,-0.978147600733808,-2.92774812072069E-17));
#123932=DIRECTION('ref_axis',(0.978147600733808,0.207911690817749,-8.19440684934305E-34));
#123933=DIRECTION('center_axis',(0.207911690817754,-0.978147600733807,0.));
#123934=DIRECTION('ref_axis',(0.978147600733807,0.207911690817754,0.));
#123935=DIRECTION('center_axis',(0.207911690817749,-0.978147600733808,-2.92774812072069E-17));
#123936=DIRECTION('ref_axis',(0.978147600733808,0.207911690817749,-3.83359069178834E-33));
#123937=DIRECTION('center_axis',(-0.207911690817754,0.978147600733807,0.));
#123938=DIRECTION('ref_axis',(-0.978147600733807,-0.207911690817754,0.));
#123939=DIRECTION('center_axis',(0.110177439185349,-0.518344097776638,-0.848045003637591));
#123940=DIRECTION('ref_axis',(1.11828009136564E-15,0.853239582811878,-0.521519140898024));
#123941=DIRECTION('center_axis',(-0.103956917928284,0.489078846173999,0.866022425483291));
#123942=DIRECTION('ref_axis',(-2.88334954178905E-16,-0.870740269393778,
0.491743208652698));
#123943=DIRECTION('center_axis',(-0.110177412160068,0.518344074628259,0.848045021297504));
#123944=DIRECTION('ref_axis',(-0.172101506936992,0.830401496087603,-0.52991926423323));
#123945=DIRECTION('center_axis',(0.110177427516376,-0.518344042878435,-0.848045038708625));
#123946=DIRECTION('ref_axis',(3.87763046936564E-16,0.85323961698728,-0.521519084984815));
#123947=DIRECTION('center_axis',(-0.103956910521019,0.489078861909796,0.866022417485797));
#123948=DIRECTION('ref_axis',(-0.175605160695512,0.848034685338496,-0.499999999999942));
#123949=DIRECTION('center_axis',(-0.180092991631446,0.84710517867207,0.499979330204955));
#123950=DIRECTION('ref_axis',(0.104894406043488,-0.488852904975612,0.86603695121957));
#123951=DIRECTION('center_axis',(0.978197989689811,0.207674488001809,-1.33614410777024E-14));
#123952=DIRECTION('ref_axis',(-0.207674488001809,0.97819798968981,1.40420698398036E-28));
#123953=DIRECTION('center_axis',(0.207911690817749,-0.978147600733808,-2.92774812072069E-17));
#123954=DIRECTION('ref_axis',(0.978147600733808,0.207911690817749,-8.19440684934305E-34));
#123955=DIRECTION('center_axis',(-0.207911690817754,0.978147600733807,0.));
#123956=DIRECTION('ref_axis',(-0.978147600733807,-0.207911690817754,0.));
#123957=DIRECTION('center_axis',(-1.70094388097117E-16,1.37739719617122E-16,
-1.));
#123958=DIRECTION('ref_axis',(-1.,7.04637109130665E-33,2.25664243350207E-16));
#123959=DIRECTION('center_axis',(0.978097154258596,0.208148881407602,0.));
#123960=DIRECTION('ref_axis',(-0.208148881407602,0.978097154258596,0.));
#123961=DIRECTION('center_axis',(-0.110177535564893,0.518344551206598,-0.848044713969303));
#123962=DIRECTION('ref_axis',(-1.36566886276548E-15,0.85323930054103,0.521519602711397));
#123963=DIRECTION('center_axis',(-0.11017742751637,0.518344042878406,0.848045038708643));
#123964=DIRECTION('ref_axis',(2.91791121664691E-16,-0.853239616987298,0.521519084984786));
#123965=DIRECTION('center_axis',(-0.110177567008161,0.518344577866136,-0.848044693589282));
#123966=DIRECTION('ref_axis',(0.171882402214125,-0.830446875605937,-0.529919264233185));
#123967=DIRECTION('center_axis',(-0.110177549147491,0.518344615107839,-0.848044673146738));
#123968=DIRECTION('ref_axis',(3.5353103468128E-15,0.853239260760973,0.5215196677941));
#123969=DIRECTION('center_axis',(0.110177412122302,-0.518344074798144,-0.848045021198573));
#123970=DIRECTION('ref_axis',(-0.180532167034328,0.828609503964605,-0.529919264233167));
#123971=DIRECTION('center_axis',(-0.110177439185351,0.518344097776645,0.848045003637586));
#123972=DIRECTION('ref_axis',(-2.03810354964487E-15,-0.853239582811873,
0.521519140898031));
#123973=DIRECTION('center_axis',(0.978201246800566,0.207659145615641,0.));
#123974=DIRECTION('ref_axis',(-0.207659145615641,0.978201246800566,0.));
#123975=DIRECTION('center_axis',(-0.207911690817754,0.978147600733807,-2.83991567709924E-15));
#123976=DIRECTION('ref_axis',(-0.978147600733807,-0.207911690817754,-8.15748401032363E-30));
#123977=DIRECTION('center_axis',(-1.70094388097117E-16,1.37739719617122E-16,
-1.));
#123978=DIRECTION('ref_axis',(-1.,-7.29277756332989E-33,1.20114286872534E-16));
#123979=DIRECTION('center_axis',(0.978093889466684,0.208164222161096,1.3360019147774E-14));
#123980=DIRECTION('ref_axis',(-0.208164222161096,0.978093889466684,3.50631737784726E-29));
#123981=DIRECTION('center_axis',(-0.207911690817749,0.978147600733808,2.92774812072069E-17));
#123982=DIRECTION('ref_axis',(-0.978147600733808,-0.207911690817749,1.87865085870298E-31));
#123983=DIRECTION('center_axis',(-0.180025927304454,0.84709989316138,-0.500012436349487));
#123984=DIRECTION('ref_axis',(-0.104926459513297,0.48887998035603,0.866017784402314));
#123985=DIRECTION('center_axis',(0.110177549147416,-0.51834461510785,0.848044673146742));
#123986=DIRECTION('ref_axis',(3.90302724780887E-15,-0.853239260760969,-0.521519667794107));
#123987=DIRECTION('center_axis',(0.103956896855725,-0.489078698391826,0.866022511471547));
#123988=DIRECTION('ref_axis',(0.184432991083765,-0.846158656399562,-0.499999999999985));
#123989=DIRECTION('center_axis',(-0.103956889752269,0.489078713616271,-0.866022503726369));
#123990=DIRECTION('ref_axis',(-1.13722082929134E-15,0.87074034548476,0.491743073916737));
#123991=DIRECTION('center_axis',(0.110177567041805,-0.518344577660503,0.848044693710599));
#123992=DIRECTION('ref_axis',(0.18075078662755,-0.828561842307535,-0.529919264233209));
#123993=DIRECTION('center_axis',(0.110177535564769,-0.518344551206596,0.848044713969321));
#123994=DIRECTION('ref_axis',(2.49956668273804E-15,-0.853239300541035,-0.521519602711388));
#123995=DIRECTION('center_axis',(-0.207911690817754,0.978147600733807,0.));
#123996=DIRECTION('ref_axis',(-0.978147600733807,-0.207911690817754,0.));
#123997=DIRECTION('center_axis',(0.207911690817757,-0.978147600733806,0.));
#123998=DIRECTION('ref_axis',(0.978147600733806,0.207911690817757,0.));
#123999=DIRECTION('center_axis',(-0.207911690817749,0.978147600733808,2.92774812072069E-17));
#124000=DIRECTION('ref_axis',(-0.978147600733808,-0.207911690817749,1.87865085870298E-31));
#124001=DIRECTION('center_axis',(-0.207911690817754,0.978147600733807,-5.67983135419817E-15));
#124002=DIRECTION('ref_axis',(-0.978147600733807,-0.207911690817754,-1.62169121129155E-29));
#124003=DIRECTION('center_axis',(-0.207911690817749,0.978147600733808,2.92774812072069E-17));
#124004=DIRECTION('ref_axis',(-0.978147600733808,-0.207911690817749,1.87865085870298E-31));
#124005=DIRECTION('center_axis',(0.180025582247342,-0.847119506978929,-0.499979330205042));
#124006=DIRECTION('ref_axis',(-0.103008581347892,0.489253749388906,-0.866036951219515));
#124007=DIRECTION('center_axis',(-0.103956917928285,0.489078846174002,0.866022425483289));
#124008=DIRECTION('ref_axis',(-6.4647814085365E-16,-0.870740269393776,0.491743208652701));
#124009=DIRECTION('center_axis',(-0.103956919795632,0.489078854959153,0.866022420297794));
#124010=DIRECTION('ref_axis',(0.978147600733986,0.207911690816909,5.24514813542623E-13));
#124011=DIRECTION('center_axis',(0.0522647557775586,-0.49726593457861,0.866022508720861));
#124012=DIRECTION('ref_axis',(-0.994521895368301,-0.10452846326739,1.39870617599167E-13));
#124013=DIRECTION('center_axis',(0.0905534316548002,-0.861270944309356,
0.500012436349347));
#124014=DIRECTION('ref_axis',(0.0512812291256691,-0.49737655014895,-0.866017784402428));
#124015=DIRECTION('center_axis',(-0.052264756681742,0.497265943181925,-0.866022503726311));
#124016=DIRECTION('ref_axis',(-9.31368434701196E-16,0.867207748104374,0.497946504785143));
#124017=DIRECTION('center_axis',(-0.104528463267628,0.994521895368276,0.));
#124018=DIRECTION('ref_axis',(-0.994521895368276,-0.104528463267628,0.));
#124019=DIRECTION('center_axis',(0.104528463267644,-0.994521895368274,-1.47193748793052E-17));
#124020=DIRECTION('ref_axis',(0.994521895368274,0.104528463267644,-6.04857834754731E-34));
#124021=DIRECTION('center_axis',(0.104528463267629,-0.994521895368276,-7.13889681646191E-16));
#124022=DIRECTION('ref_axis',(0.994521895368276,0.104528463267629,5.1828952049124E-31));
#124023=DIRECTION('center_axis',(0.104528463267644,-0.994521895368274,-1.47193748793052E-17));
#124024=DIRECTION('ref_axis',(0.994521895368274,0.104528463267644,-3.02439851631779E-35));
#124025=DIRECTION('center_axis',(-0.10452846326763,0.994521895368276,0.));
#124026=DIRECTION('ref_axis',(-0.994521895368276,-0.10452846326763,0.));
#124027=DIRECTION('center_axis',(0.0553921636609794,-0.527021232978627,
-0.848045003637568));
#124028=DIRECTION('ref_axis',(-1.03878386976432E-15,0.849349030019369,-0.527831625809933));
#124029=DIRECTION('center_axis',(-0.0522647708473857,0.497266077958573,
0.866022425483295));
#124030=DIRECTION('ref_axis',(4.0027550172051E-16,-0.867207670398082,0.497946640115919));
#124031=DIRECTION('center_axis',(-0.0553921391978153,0.52702120713269,0.848045021297509));
#124032=DIRECTION('ref_axis',(-0.084358124572687,0.843841975853974,-0.529919264233185));
#124033=DIRECTION('center_axis',(0.0553921577943494,-0.527021177161371,
-0.848045038708634));
#124034=DIRECTION('ref_axis',(1.11869826565349E-15,0.849349064867504,-0.527831569734793));
#124035=DIRECTION('center_axis',(-0.052264761841082,0.497266092833372,0.866022417485788));
#124036=DIRECTION('ref_axis',(-0.0859994148082359,0.861744800188948,-0.499999999999951));
#124037=DIRECTION('center_axis',(-0.0905598208270846,0.861289491529776,
0.499979330204906));
#124038=DIRECTION('ref_axis',(0.0532207405856546,-0.497139368682233,0.866036951219603));
#124039=DIRECTION('center_axis',(0.994547213842469,0.104287292793425,-1.35847590536994E-14));
#124040=DIRECTION('ref_axis',(-0.104287292793425,0.994547213842469,7.25153974882784E-30));
#124041=DIRECTION('center_axis',(0.104528463267644,-0.994521895368274,-1.47193748793052E-17));
#124042=DIRECTION('ref_axis',(0.994521895368274,0.104528463267644,-6.04857834754731E-34));
#124043=DIRECTION('center_axis',(-0.104528463267628,0.994521895368276,0.));
#124044=DIRECTION('ref_axis',(-0.994521895368276,-0.104528463267628,0.));
#124045=DIRECTION('center_axis',(-1.55536281769216E-16,1.40045497140052E-16,
-1.));
#124046=DIRECTION('ref_axis',(-1.,-6.26344097005036E-33,1.12832121675104E-16));
#124047=DIRECTION('center_axis',(0.994496518411992,0.104769627595152,0.));
#124048=DIRECTION('ref_axis',(-0.104769627595152,0.994496518411992,0.));
#124049=DIRECTION('center_axis',(-0.055392212116204,0.527021693999018,-0.848044713969304));
#124050=DIRECTION('ref_axis',(8.65376607539225E-16,0.849348742192389,0.527832088960312));
#124051=DIRECTION('center_axis',(-0.0553921577943474,0.527021177161352,
0.848045038708646));
#124052=DIRECTION('ref_axis',(1.30911556478354E-16,-0.849349064867516,0.527831569734774));
#124053=DIRECTION('center_axis',(-0.0553922406001646,0.527021723799264,
-0.848044693589286));
#124054=DIRECTION('ref_axis',(0.0841354767040651,-0.843864204095861,-0.529919264233183));
#124055=DIRECTION('center_axis',(-0.0553922189449436,0.527021758969971,
-0.848044673146736));
#124056=DIRECTION('ref_axis',(-1.08455201048859E-15,0.849348701629311,0.527832154231441));
#124057=DIRECTION('center_axis',(0.0553921391498299,-0.527021207296933,
-0.848045021198574));
#124058=DIRECTION('ref_axis',(-0.0929299148210875,0.842941044395081,-0.529919264233218));
#124059=DIRECTION('center_axis',(-0.0553921636609763,0.527021232978597,
0.848045003637587));
#124060=DIRECTION('ref_axis',(-1.18714675169444E-15,-0.849349030019387,
0.527831625809904));
#124061=DIRECTION('center_axis',(0.994548849394384,0.104271693993661,-1.09530233639679E-15));
#124062=DIRECTION('ref_axis',(-0.104271693993661,0.994548849394384,-4.94221831143587E-30));
#124063=DIRECTION('center_axis',(-0.104528463267629,0.994521895368276,0.));
#124064=DIRECTION('ref_axis',(-0.994521895368276,-0.104528463267629,0.));
#124065=DIRECTION('center_axis',(-1.55536281769216E-16,1.40045497140052E-16,
-1.));
#124066=DIRECTION('ref_axis',(-1.,-5.41749190418792E-33,1.20114286872534E-16));
#124067=DIRECTION('center_axis',(0.99449487505034,0.104785225574074,0.));
#124068=DIRECTION('ref_axis',(-0.104785225574074,0.994494875050339,0.));
#124069=DIRECTION('center_axis',(-0.104528463267644,0.994521895368274,1.47193748793052E-17));
#124070=DIRECTION('ref_axis',(-0.994521895368274,-0.104528463267644,-2.00812407505412E-32));
#124071=DIRECTION('center_axis',(-0.090493676371101,0.861277224842662,-0.500012436349501));
#124072=DIRECTION('ref_axis',(-0.0532497883198399,0.49716964624041,0.866017784402305));
#124073=DIRECTION('center_axis',(0.0553922189448982,-0.527021758969983,
0.848044673146731));
#124074=DIRECTION('ref_axis',(3.68113899431711E-16,-0.849348701629304,-0.527832154231452));
#124075=DIRECTION('center_axis',(0.0522647653332842,-0.497265928783765,
0.866022511471541));
#124076=DIRECTION('ref_axis',(0.0949749838225286,-0.860801807879101,-0.499999999999982));
#124077=DIRECTION('center_axis',(-0.0522647566817781,0.49726594318182,-0.86602250372637));
#124078=DIRECTION('ref_axis',(5.50301678318796E-16,0.867207748104434,0.497946504785038));
#124079=DIRECTION('center_axis',(0.0553922406592559,-0.527021723597822,
0.848044693710613));
#124080=DIRECTION('ref_axis',(0.0931523188204474,-0.842916495800706,-0.529919264233177));
#124081=DIRECTION('center_axis',(0.0553922121161434,-0.527021693999,0.848044713969319));
#124082=DIRECTION('ref_axis',(4.25528683943419E-16,-0.849348742192401,-0.527832088960292));
#124083=DIRECTION('center_axis',(-0.104528463267629,0.994521895368276,-7.1388968164623E-16));
#124084=DIRECTION('ref_axis',(-0.994521895368276,-0.104528463267629,5.0770299838595E-31));
#124085=DIRECTION('center_axis',(0.104528463267629,-0.994521895368276,0.));
#124086=DIRECTION('ref_axis',(0.994521895368276,0.104528463267629,0.));
#124087=DIRECTION('center_axis',(-0.104528463267644,0.994521895368274,1.47193748793052E-17));
#124088=DIRECTION('ref_axis',(-0.994521895368274,-0.104528463267644,-2.00812407505412E-32));
#124089=DIRECTION('center_axis',(-0.104528463267629,0.994521895368276,0.));
#124090=DIRECTION('ref_axis',(-0.994521895368276,-0.104528463267629,0.));
#124091=DIRECTION('center_axis',(-0.104528463267644,0.994521895368274,1.47193748793052E-17));
#124092=DIRECTION('ref_axis',(-0.994521895368274,-0.104528463267644,-2.00812407505412E-32));
#124093=DIRECTION('center_axis',(0.0904912830029371,-0.861296695145102,
-0.499979330205368));
#124094=DIRECTION('ref_axis',(-0.0513033469792888,0.497340894871386,-0.866036951219318));
#124095=DIRECTION('center_axis',(-0.0522647708473827,0.497266077958545,
0.866022425483311));
#124096=DIRECTION('ref_axis',(-3.47519388666402E-16,-0.867207670398098,
0.49794664011589));
#124097=DIRECTION('center_axis',(-0.0522647717850455,0.497266086879728,
0.86602242030422));
#124098=DIRECTION('ref_axis',(0.99452189536868,0.104528463263786,2.23792987110329E-12));
#124099=DIRECTION('center_axis',(-5.08727263162943E-15,-0.500005014362422,
0.866022508721589));
#124100=DIRECTION('ref_axis',(-1.,-7.55301335024474E-12,-4.33598914551087E-12));
#124101=DIRECTION('center_axis',(3.00422138958798E-5,-0.866018223016285,
0.500012436346518));
#124102=DIRECTION('ref_axis',(-0.00098970131624398,-0.500012217437995,-0.866017784404017));
#124103=DIRECTION('center_axis',(-2.73187543788774E-14,0.500005023014372,
-0.866022503726316));
#124104=DIRECTION('ref_axis',(-3.29182907633956E-28,0.866022503726316,0.500005023014372));
#124105=DIRECTION('center_axis',(0.,1.,0.));
#124106=DIRECTION('ref_axis',(0.,0.,1.));
#124107=DIRECTION('center_axis',(-1.04744440165294E-14,-1.,1.4749788077992E-30));
#124108=DIRECTION('ref_axis',(1.,-1.04744440165294E-14,-2.48920611114446E-60));
#124109=DIRECTION('center_axis',(0.,-1.,0.));
#124110=DIRECTION('ref_axis',(0.,0.,-1.));
#124111=DIRECTION('center_axis',(-1.04744440165294E-14,-1.,1.4749788077992E-30));
#124112=DIRECTION('ref_axis',(1.,-1.04744440165294E-14,-2.48920611114446E-60));
#124113=DIRECTION('center_axis',(0.,1.,0.));
#124114=DIRECTION('ref_axis',(0.,0.,1.));
#124115=DIRECTION('center_axis',(0.,-0.52992421326579,-0.848045003637563));
#124116=DIRECTION('ref_axis',(0.,0.848045003637563,-0.52992421326579));
#124117=DIRECTION('center_axis',(0.,0.500005158533422,0.866022425483294));
#124118=DIRECTION('ref_axis',(0.,-0.866022425483294,0.500005158533421));
#124119=DIRECTION('center_axis',(2.16240926169255E-8,0.529924185004365,
0.84804502129749));
#124120=DIRECTION('ref_axis',(0.00430950301662301,0.848037146343398,-0.529919264233237));
#124121=DIRECTION('center_axis',(0.,-0.529924157141051,-0.848045038708645));
#124122=DIRECTION('ref_axis',(0.,0.848045038708645,-0.529924157141051));
#124123=DIRECTION('center_axis',(1.05144329133207E-8,0.500005172385368,
0.866022417485759));
#124124=DIRECTION('ref_axis',(0.00454855868433578,0.866013458679421,-0.500000000000001));
#124125=DIRECTION('center_axis',(-3.44576744524761E-5,0.866037336481559,
0.499979330205355));
#124126=DIRECTION('ref_axis',(0.000963977578947313,-0.499979069431867,0.866036951219329));
#124127=DIRECTION('center_axis',(-1.04744440165294E-14,-1.,1.4749788077992E-30));
#124128=DIRECTION('ref_axis',(1.,-1.04744440165294E-14,-2.48920611114446E-60));
#124129=DIRECTION('center_axis',(0.,1.,0.));
#124130=DIRECTION('ref_axis',(0.,0.,1.));
#124131=DIRECTION('center_axis',(-2.89534733035821E-14,0.529924676825566,
-0.848044713969328));
#124132=DIRECTION('ref_axis',(-3.84874727475395E-28,0.848044713969328,0.529924676825566));
#124133=DIRECTION('center_axis',(0.,0.529924157141041,0.848045038708651));
#124134=DIRECTION('ref_axis',(0.,-0.848045038708651,0.529924157141041));
#124135=DIRECTION('center_axis',(-2.52137135654268E-8,0.529924709439987,
-0.848044693589285));
#124136=DIRECTION('ref_axis',(-0.00453325468848542,-0.848035979777079,-0.529919264233202));
#124137=DIRECTION('center_axis',(-4.63345827774717E-14,0.529924742154432,
-0.848044673146739));
#124138=DIRECTION('ref_axis',(-1.03401629657842E-27,0.848044673146739,0.529924742154432));
#124139=DIRECTION('center_axis',(-2.16959060264487E-8,-0.529924185162668,
-0.848045021198569));
#124140=DIRECTION('ref_axis',(-0.00430950303050303,0.848037146343343,-0.529919264233213));
#124141=DIRECTION('center_axis',(0.,0.52992421326579,0.848045003637563));
#124142=DIRECTION('ref_axis',(0.,-0.848045003637563,0.52992421326579));
#124143=DIRECTION('center_axis',(0.,1.,0.));
#124144=DIRECTION('ref_axis',(0.,0.,1.));
#124145=DIRECTION('center_axis',(1.04744440165294E-14,1.,-1.4749788077992E-30));
#124146=DIRECTION('ref_axis',(-1.,1.04744440165294E-14,-2.83769496670468E-58));
#124147=DIRECTION('center_axis',(3.00422154286595E-5,0.866018223015636,
-0.500012436347643));
#124148=DIRECTION('ref_axis',(-0.000989701290563527,0.500012217439134,0.86601778440339));
#124149=DIRECTION('center_axis',(0.,-0.529924742154432,0.848044673146739));
#124150=DIRECTION('ref_axis',(0.,-0.848044673146739,-0.529924742154432));
#124151=DIRECTION('center_axis',(1.01107237965894E-8,-0.500005009599421,
0.866022511471545));
#124152=DIRECTION('ref_axis',(0.00447641076555513,-0.866013834616201,-0.500000000000002));
#124153=DIRECTION('center_axis',(0.,0.500005023014355,-0.866022503726326));
#124154=DIRECTION('ref_axis',(0.,0.866022503726326,0.500005023014355));
#124155=DIRECTION('center_axis',(2.52897127115498E-8,-0.529924709245837,
0.848044693710606));
#124156=DIRECTION('ref_axis',(0.00453325469237332,-0.848035979777063,-0.529919264233195));
#124157=DIRECTION('center_axis',(-2.89534733035821E-14,-0.529924676825566,
0.848044713969328));
#124158=DIRECTION('ref_axis',(-3.89468630110175E-28,-0.848044713969328,
-0.529924676825566));
#124159=DIRECTION('center_axis',(0.,1.,0.));
#124160=DIRECTION('ref_axis',(0.,0.,1.));
#124161=DIRECTION('center_axis',(0.,-1.,0.));
#124162=DIRECTION('ref_axis',(0.,0.,-1.));
#124163=DIRECTION('center_axis',(1.04744440165294E-14,1.,-1.4749788077992E-30));
#124164=DIRECTION('ref_axis',(-1.,1.04744440165294E-14,-2.83769496670468E-58));
#124165=DIRECTION('center_axis',(0.,1.,0.));
#124166=DIRECTION('ref_axis',(0.,0.,1.));
#124167=DIRECTION('center_axis',(1.04744440165294E-14,1.,-1.4749788077992E-30));
#124168=DIRECTION('ref_axis',(-1.,1.04744440165294E-14,-2.83769496670468E-58));
#124169=DIRECTION('center_axis',(-3.44576745143992E-5,-0.866037336481586,
-0.499979330205309));
#124170=DIRECTION('ref_axis',(0.000963977574060321,0.499979069431824,-0.86603695121936));
#124171=DIRECTION('center_axis',(0.,0.500005158533422,0.866022425483294));
#124172=DIRECTION('ref_axis',(0.,-0.866022425483294,0.500005158533422));
#124173=DIRECTION('center_axis',(5.43769792106264E-15,0.500005167509914,
0.866022420300643));
#124174=DIRECTION('ref_axis',(1.,-1.67844740333718E-12,9.44126664377163E-13));
#124175=DIRECTION('center_axis',(-0.0522647557773824,-0.497265934576869,
0.866022508721871));
#124176=DIRECTION('ref_axis',(-0.994521895368246,0.104528463267908,1.39870617597895E-13));
#124177=DIRECTION('center_axis',(-0.0904936763721428,-0.861277224842625,
0.500012436349377));
#124178=DIRECTION('ref_axis',(-0.0532497883297758,-0.497169646239235,-0.866017784402369));
#124179=DIRECTION('center_axis',(0.0522647566817887,0.497265943181924,-0.866022503726309));
#124180=DIRECTION('ref_axis',(9.3445928215498E-16,0.867207748104374,0.497946504785143));
#124181=DIRECTION('center_axis',(0.104528463267683,0.99452189536827,0.));
#124182=DIRECTION('ref_axis',(-0.99452189536827,0.104528463267683,0.));
#124183=DIRECTION('center_axis',(-0.104528463267664,-0.994521895368272,
1.4719374879308E-17));
#124184=DIRECTION('ref_axis',(0.994521895368272,-0.104528463267664,7.55090158384622E-35));
#124185=DIRECTION('center_axis',(-0.104528463267683,-0.99452189536827,0.));
#124186=DIRECTION('ref_axis',(0.99452189536827,-0.104528463267683,0.));
#124187=DIRECTION('center_axis',(-0.104528463267664,-0.994521895368272,
1.4719374879308E-17));
#124188=DIRECTION('ref_axis',(0.994521895368272,-0.104528463267664,-4.99104833753089E-34));
#124189=DIRECTION('center_axis',(0.104528463267682,0.994521895368271,0.));
#124190=DIRECTION('ref_axis',(-0.994521895368271,0.104528463267682,0.));
#124191=DIRECTION('center_axis',(-0.055392163661009,-0.527021232978633,
-0.848045003637563));
#124192=DIRECTION('ref_axis',(5.85670520831155E-16,0.849349030019364,-0.52783162580994));
#124193=DIRECTION('center_axis',(0.052264770847414,0.497266077958582,0.866022425483288));
#124194=DIRECTION('ref_axis',(1.6088847247092E-16,-0.867207670398076,0.497946640115928));
#124195=DIRECTION('center_axis',(0.0553921822216235,0.527021202610695,0.848045021297516));
#124196=DIRECTION('ref_axis',(0.0929299148295972,0.842941044394173,-0.52991926423317));
#124197=DIRECTION('center_axis',(-0.0553921577943759,-0.527021177161348,
-0.848045038708647));
#124198=DIRECTION('ref_axis',(3.66225041260374E-16,0.849349064867518,-0.527831569734771));
#124199=DIRECTION('center_axis',(0.0522647827539146,0.497266090635403,0.866022417485754));
#124200=DIRECTION('ref_axis',(0.0950466972136718,0.860793892490397,-0.500000000000004));
#124201=DIRECTION('center_axis',(0.0904912830033326,0.861296695144991,0.499979330205487));
#124202=DIRECTION('ref_axis',(-0.0513033469766535,-0.497340894871782,0.866036951219247));
#124203=DIRECTION('center_axis',(0.994496518411991,-0.104769627595163,6.79203329632462E-15));
#124204=DIRECTION('ref_axis',(0.104769627595163,0.994496518411991,2.96919234963523E-30));
#124205=DIRECTION('center_axis',(-0.104528463267664,-0.994521895368272,
1.4719374879308E-17));
#124206=DIRECTION('ref_axis',(0.994521895368272,-0.104528463267664,7.55090158384622E-35));
#124207=DIRECTION('center_axis',(0.104528463267628,0.994521895368276,0.));
#124208=DIRECTION('ref_axis',(-0.994521895368276,0.104528463267628,0.));
#124209=DIRECTION('center_axis',(-1.26097532010602E-16,1.40045497140051E-16,
-1.));
#124210=DIRECTION('ref_axis',(0.,1.,1.12832121675104E-16));
#124211=DIRECTION('center_axis',(0.994547213842467,-0.104287292793444,0.));
#124212=DIRECTION('ref_axis',(0.104287292793444,0.994547213842467,0.));
#124213=DIRECTION('center_axis',(0.0553922121162013,0.527021693998993,-0.84804471396932));
#124214=DIRECTION('ref_axis',(7.93731044687634E-16,0.849348742192405,0.527832088960286));
#124215=DIRECTION('center_axis',(0.0553921577943754,0.527021177161343,0.84804503870865));
#124216=DIRECTION('ref_axis',(-6.93579166402575E-16,-0.849349064867522,
0.527831569734766));
#124217=DIRECTION('center_axis',(0.0553921904558474,0.52702172906962,-0.848044693589301));
#124218=DIRECTION('ref_axis',(-0.0931523188100742,-0.842916495801844,-0.529919264233191));
#124219=DIRECTION('center_axis',(0.0553922189449272,0.527021758969979,-0.848044673146731));
#124220=DIRECTION('ref_axis',(5.64549624567747E-16,0.849348701629306,0.527832154231449));
#124221=DIRECTION('center_axis',(-0.0553921822949527,-0.527021202762207,
-0.848045021198568));
#124222=DIRECTION('ref_axis',(0.0843581245765446,0.843841975853581,-0.529919264233197));
#124223=DIRECTION('center_axis',(0.0553921636610064,0.527021232978609,0.848045003637578));
#124224=DIRECTION('ref_axis',(-5.90605431002811E-16,-0.84934903001938,0.527831625809916));
#124225=DIRECTION('center_axis',(0.994494875050337,-0.104785225574097,-1.06687590778408E-15));
#124226=DIRECTION('ref_axis',(0.104785225574097,0.994494875050337,3.46902153471063E-31));
#124227=DIRECTION('center_axis',(0.104528463267683,0.99452189536827,7.1388968164656E-16));
#124228=DIRECTION('ref_axis',(-0.99452189536827,0.104528463267683,2.13048964590254E-33));
#124229=DIRECTION('center_axis',(-1.26097532010602E-16,1.40045497140051E-16,
-1.));
#124230=DIRECTION('ref_axis',(0.,1.,1.20114286872534E-16));
#124231=DIRECTION('center_axis',(0.994548849394382,-0.104271693993677,1.0953023363959E-15));
#124232=DIRECTION('ref_axis',(0.104271693993677,0.994548849394382,-2.25165513859667E-30));
#124233=DIRECTION('center_axis',(0.104528463267664,0.994521895368272,-1.4719374879308E-17));
#124234=DIRECTION('ref_axis',(-0.994521895368272,0.104528463267664,-1.2142399857261E-32));
#124235=DIRECTION('center_axis',(0.0905534316547619,0.861270944309424,-0.500012436349237));
#124236=DIRECTION('ref_axis',(0.0512812291215075,0.497376550149274,0.866017784402488));
#124237=DIRECTION('center_axis',(-0.0553922189449268,-0.527021758969972,
0.848044673146736));
#124238=DIRECTION('ref_axis',(-1.04823533788178E-15,-0.84934870162931,-0.527832154231442));
#124239=DIRECTION('center_axis',(-0.0522647452196774,-0.49726593089775,
0.866022511471565));
#124240=DIRECTION('ref_axis',(-0.0860712067697641,-0.861737632557173,-0.499999999999955));
#124241=DIRECTION('center_axis',(0.0522647566818046,0.497265943181812,-0.866022503726373));
#124242=DIRECTION('ref_axis',(-1.28065569756335E-16,0.867207748104438,0.497946504785031));
#124243=DIRECTION('center_axis',(-0.055392190356225,-0.527021728884907,
0.848044693710599));
#124244=DIRECTION('ref_axis',(-0.0841354767102596,-0.843864204095235,-0.529919264233197));
#124245=DIRECTION('center_axis',(-0.0553922121162459,-0.527021693998973,
0.848044713969329));
#124246=DIRECTION('ref_axis',(-3.6090586595327E-16,-0.849348742192416,-0.527832088960269));
#124247=DIRECTION('center_axis',(0.104528463267683,0.99452189536827,-5.36237632086923E-14));
#124248=DIRECTION('ref_axis',(-0.99452189536827,0.104528463267683,5.67004406102361E-31));
#124249=DIRECTION('center_axis',(-0.104528463267684,-0.99452189536827,0.));
#124250=DIRECTION('ref_axis',(0.99452189536827,-0.104528463267684,0.));
#124251=DIRECTION('center_axis',(0.104528463267664,0.994521895368272,-1.4719374879308E-17));
#124252=DIRECTION('ref_axis',(-0.994521895368272,0.104528463267664,-1.2142399857261E-32));
#124253=DIRECTION('center_axis',(0.104528463267683,0.99452189536827,9.28056586140528E-15));
#124254=DIRECTION('ref_axis',(-0.99452189536827,0.104528463267683,2.74937968383573E-32));
#124255=DIRECTION('center_axis',(0.104528463267664,0.994521895368272,-1.4719374879308E-17));
#124256=DIRECTION('ref_axis',(-0.994521895368272,0.104528463267664,-1.2142399857261E-32));
#124257=DIRECTION('center_axis',(-0.0905598208270262,-0.861289491529606,
-0.49997933020521));
#124258=DIRECTION('ref_axis',(0.0532207406056314,0.497139368680429,-0.866036951219411));
#124259=DIRECTION('center_axis',(0.0522647708474102,0.497266077958546,0.866022425483309));
#124260=DIRECTION('ref_axis',(4.84777660203887E-16,-0.867207670398097,0.497946640115892));
#124261=DIRECTION('center_axis',(0.0522647717852642,0.497266086881686,0.866022420303083));
#124262=DIRECTION('ref_axis',(0.994521895367867,-0.104528463271519,2.23792987111612E-12));
#124263=DIRECTION('center_axis',(-0.103956887952481,-0.489078705148897,
0.86602250872429));
#124264=DIRECTION('ref_axis',(-0.978147600733677,0.207911690818365,3.49676543997127E-13));
#124265=DIRECTION('center_axis',(-0.180025927304388,-0.847099893162094,
0.500012436348302));
#124266=DIRECTION('ref_axis',(-0.104926459550624,-0.488879980346867,-0.866017784402964));
#124267=DIRECTION('center_axis',(0.103956889752339,0.489078713616364,-0.866022503726308));
#124268=DIRECTION('ref_axis',(2.29104531904658E-15,0.870740345484705,0.491743073916834));
#124269=DIRECTION('center_axis',(0.207911690817757,0.978147600733806,5.62829268885415E-14));
#124270=DIRECTION('ref_axis',(-0.978147600733806,0.207911690817757,-6.75602897704988E-32));
#124271=DIRECTION('center_axis',(-0.20791169081777,-0.978147600733803,2.92774812072098E-17));
#124272=DIRECTION('ref_axis',(0.978147600733803,-0.20791169081777,9.03770998686543E-34));
#124273=DIRECTION('center_axis',(-0.207911690817757,-0.978147600733806,
-2.83991567709912E-15));
#124274=DIRECTION('ref_axis',(0.978147600733806,-0.207911690817757,-1.96908327204163E-32));
#124275=DIRECTION('center_axis',(-0.20791169081777,-0.978147600733803,2.92774812072098E-17));
#124276=DIRECTION('ref_axis',(0.978147600733803,-0.20791169081777,-1.35684150645397E-33));
#124277=DIRECTION('center_axis',(0.207911690817754,0.978147600733807,0.));
#124278=DIRECTION('ref_axis',(-0.978147600733807,0.207911690817754,0.));
#124279=DIRECTION('center_axis',(-0.110177439185351,-0.518344097776641,
-0.848045003637589));
#124280=DIRECTION('ref_axis',(-1.51970787343667E-15,0.853239582811876,-0.521519140898027));
#124281=DIRECTION('center_axis',(0.103956917928287,0.489078846173999,0.866022425483291));
#124282=DIRECTION('ref_axis',(2.96906041204586E-16,-0.870740269393778,0.491743208652698));
#124283=DIRECTION('center_axis',(0.110177454466897,0.518344065635659,0.848045021297508));
#124284=DIRECTION('ref_axis',(0.180532167028516,0.828609503965844,-0.52991926423321));
#124285=DIRECTION('center_axis',(-0.110177427516368,-0.51834404287839,-0.848045038708654));
#124286=DIRECTION('ref_axis',(-2.67094448372999E-15,0.853239616987309,-0.521519084984769));
#124287=DIRECTION('center_axis',(0.103956931095903,0.489078857536534,0.86602241748576));
#124288=DIRECTION('ref_axis',(0.18450348422679,0.846143288284058,-0.500000000000016));
#124289=DIRECTION('center_axis',(0.18002558224756,0.847119506978716,0.499979330205324));
#124290=DIRECTION('ref_axis',(-0.103008581357447,-0.489253749387169,0.86603695121936));
#124291=DIRECTION('center_axis',(0.978097154258593,-0.208148881407615,0.));
#124292=DIRECTION('ref_axis',(0.208148881407615,0.978097154258593,0.));
#124293=DIRECTION('center_axis',(-0.20791169081777,-0.978147600733803,2.92774812072098E-17));
#124294=DIRECTION('ref_axis',(0.978147600733803,-0.20791169081777,9.03770998686543E-34));
#124295=DIRECTION('center_axis',(0.207911690817809,0.978147600733795,0.));
#124296=DIRECTION('ref_axis',(-0.978147600733795,0.207911690817809,0.));
#124297=DIRECTION('center_axis',(-1.11539425682701E-16,1.37739719617121E-16,
-1.));
#124298=DIRECTION('ref_axis',(0.,1.,1.12832121675104E-16));
#124299=DIRECTION('center_axis',(0.978197989689803,-0.207674488001846,0.));
#124300=DIRECTION('ref_axis',(0.207674488001846,0.978197989689803,0.));
#124301=DIRECTION('center_axis',(0.110177535564859,0.518344551206574,-0.848044713969323));
#124302=DIRECTION('ref_axis',(-4.00339603515207E-16,0.853239300541046,0.521519602711371));
#124303=DIRECTION('center_axis',(0.110177427516366,0.518344042878381,0.848045038708659));
#124304=DIRECTION('ref_axis',(1.58984749529623E-15,-0.853239616987314,0.521519084984761));
#124305=DIRECTION('center_axis',(0.110177517684597,0.518344588350194,-0.848044693589276));
#124306=DIRECTION('ref_axis',(-0.18075078663936,-0.828561842304951,-0.529919264233221));
#124307=DIRECTION('center_axis',(0.110177549147491,0.518344615107832,-0.848044673146743));
#124308=DIRECTION('ref_axis',(-2.64002787776822E-15,0.853239260760977,0.521519667794094));
#124309=DIRECTION('center_axis',(-0.110177454555387,-0.518344065778716,
-0.848045021198572));
#124310=DIRECTION('ref_axis',(0.172101506935008,0.830401496088012,-0.529919264233233));
#124311=DIRECTION('center_axis',(0.110177439185354,0.518344097776652,0.848045003637582));
#124312=DIRECTION('ref_axis',(2.89201529937556E-15,-0.853239582811869,0.521519140898038));
#124313=DIRECTION('center_axis',(0.978093889466681,-0.20816422216111,-1.53465780422786E-14));
#124314=DIRECTION('ref_axis',(0.20816422216111,0.978093889466681,2.32253611591275E-29));
#124315=DIRECTION('center_axis',(0.207911690817757,0.978147600733806,5.34430112114423E-14));
#124316=DIRECTION('ref_axis',(-0.978147600733806,0.207911690817757,1.19680266142653E-30));
#124317=DIRECTION('center_axis',(-1.11539425682701E-16,1.37739719617121E-16,
-1.));
#124318=DIRECTION('ref_axis',(0.,1.,1.20114286872534E-16));
#124319=DIRECTION('center_axis',(0.978201246800563,-0.207659145615657,2.0156211610367E-15));
#124320=DIRECTION('ref_axis',(0.207659145615657,0.978201246800563,-8.63903528825318E-30));
#124321=DIRECTION('center_axis',(0.20791169081777,0.978147600733803,-2.92774812072098E-17));
#124322=DIRECTION('ref_axis',(-0.978147600733803,0.20791169081777,-1.37139085278161E-32));
#124323=DIRECTION('center_axis',(0.180084698748564,0.847087400905278,-0.500012436349517));
#124324=DIRECTION('ref_axis',(0.102990311599707,0.489291521299458,0.866017784402293));
#124325=DIRECTION('center_axis',(-0.110177549147563,-0.518344615107823,
0.848044673146739));
#124326=DIRECTION('ref_axis',(1.94829734210075E-15,-0.85323926076098,-0.521519667794088));
#124327=DIRECTION('center_axis',(-0.103956877077249,-0.489078702595896,
0.866022511471533));
#124328=DIRECTION('ref_axis',(-0.175675810178078,-0.84802005266283,-0.500000000000007));
#124329=DIRECTION('center_axis',(0.103956889752269,0.489078713616261,-0.866022503726375));
#124330=DIRECTION('ref_axis',(2.38114632574082E-15,0.870740345484765,0.491743073916727));
#124331=DIRECTION('center_axis',(-0.110177517568077,-0.51834458817644,0.848044693710616));
#124332=DIRECTION('ref_axis',(-0.171882402228799,-0.830446875602875,-0.529919264233223));
#124333=DIRECTION('center_axis',(-0.110177535564811,-0.518344551206572,
0.84804471396933));
#124334=DIRECTION('ref_axis',(-1.96158023811665E-16,-0.853239300541049,
-0.521519602711367));
#124335=DIRECTION('center_axis',(0.207911690817757,0.978147600733806,5.34430112114423E-14));
#124336=DIRECTION('ref_axis',(-0.978147600733806,0.207911690817757,1.19680266142653E-30));
#124337=DIRECTION('center_axis',(-0.207911690817757,-0.978147600733806,
0.));
#124338=DIRECTION('ref_axis',(0.978147600733806,-0.207911690817757,0.));
#124339=DIRECTION('center_axis',(0.20791169081777,0.978147600733803,-2.92774812072098E-17));
#124340=DIRECTION('ref_axis',(-0.978147600733803,0.20791169081777,-1.37139085278161E-32));
#124341=DIRECTION('center_axis',(0.207911690817757,0.978147600733806,-7.33224209511362E-14));
#124342=DIRECTION('ref_axis',(-0.978147600733806,0.207911690817757,-2.34871055257466E-31));
#124343=DIRECTION('center_axis',(0.20791169081777,0.978147600733803,-2.92774812072098E-17));
#124344=DIRECTION('ref_axis',(-0.978147600733803,0.20791169081777,-1.37139085278161E-32));
#124345=DIRECTION('center_axis',(-0.180092991631147,-0.847105178672085,
-0.499979330205039));
#124346=DIRECTION('ref_axis',(0.104894406044029,0.488852904975583,-0.866036951219522));
#124347=DIRECTION('center_axis',(0.103956917928286,0.489078846173998,0.866022425483291));
#124348=DIRECTION('ref_axis',(2.529180872252E-16,-0.870740269393778,0.491743208652698));
#124349=DIRECTION('center_axis',(0.10395691979444,0.489078854953561,0.866022420301095));
#124350=DIRECTION('ref_axis',(0.978147600733799,-0.207911690817788,3.49676542358288E-14));
#124351=DIRECTION('center_axis',(-0.154510046710454,-0.475533027088933,
0.866022508722013));
#124352=DIRECTION('ref_axis',(-0.9510565162939,0.309016994378807,2.34283284479982E-12));
#124353=DIRECTION('center_axis',(-0.267585776504412,-0.823641557783639,
0.500012436349609));
#124354=DIRECTION('ref_axis',(-0.155453534429849,-0.475234043111657,-0.866017784402269));
#124355=DIRECTION('center_axis',(0.154510049384266,0.475533035318147,-0.866022503726308));
#124356=DIRECTION('ref_axis',(-4.94155540489305E-15,0.876548788012433,0.481313018974072));
#124357=DIRECTION('center_axis',(0.309016994374964,0.951056516295148,0.));
#124358=DIRECTION('ref_axis',(-0.951056516295148,0.309016994374964,0.));
#124359=DIRECTION('center_axis',(-0.309016994374957,-0.95105651629515,4.35148173242984E-17));
#124360=DIRECTION('ref_axis',(0.95105651629515,-0.309016994374957,3.82078699478083E-35));
#124361=DIRECTION('center_axis',(-0.309016994374964,-0.951056516295148,
0.));
#124362=DIRECTION('ref_axis',(0.951056516295148,-0.309016994374964,0.));
#124363=DIRECTION('center_axis',(-0.309016994374957,-0.95105651629515,4.35148173242984E-17));
#124364=DIRECTION('ref_axis',(0.95105651629515,-0.309016994374957,3.82078699478083E-35));
#124365=DIRECTION('center_axis',(0.309016994374914,0.951056516295165,0.));
#124366=DIRECTION('ref_axis',(-0.951056516295164,0.309016994374914,0.));
#124367=DIRECTION('center_axis',(-0.163755587629897,-0.503987876168966,
-0.848045003637591));
#124368=DIRECTION('ref_axis',(2.74983269065662E-16,0.8596494620415,-0.510884333691845));
#124369=DIRECTION('center_axis',(0.154510091262001,0.47553316420445,0.866022425483262));
#124370=DIRECTION('ref_axis',(-1.17478566960452E-15,-0.876548714628813,
0.481313152617478));
#124371=DIRECTION('center_axis',(0.163755599457083,0.503987842610314,0.848045021297486));
#124372=DIRECTION('ref_axis',(0.26615647102241,0.805199544415818,-0.5299192642332));
#124373=DIRECTION('center_axis',(-0.163755570286403,-0.503987822791179,
-0.848045038708665));
#124374=DIRECTION('ref_axis',(6.13898415849569E-16,0.859649495083718,-0.510884278092709));
#124375=DIRECTION('center_axis',(0.154510105546379,0.475533174127907,0.866022417485762));
#124376=DIRECTION('ref_axis',(0.271938812471266,0.822222161141207,-0.5));
#124377=DIRECTION('center_axis',(0.267587483540056,0.823661100222809,0.499979330205211));
#124378=DIRECTION('ref_axis',(-0.153585232141186,-0.475806237444091,0.866036951219424));
#124379=DIRECTION('center_axis',(0.950981553003154,-0.309247612517397,0.));
#124380=DIRECTION('ref_axis',(0.309247612517397,0.950981553003154,0.));
#124381=DIRECTION('center_axis',(-0.309016994374957,-0.95105651629515,4.35148173242984E-17));
#124382=DIRECTION('ref_axis',(0.95105651629515,-0.309016994374957,3.82078699478083E-35));
#124383=DIRECTION('center_axis',(0.309016994374964,0.951056516295148,0.));
#124384=DIRECTION('ref_axis',(-0.951056516295148,0.309016994374964,0.));
#124385=DIRECTION('center_axis',(-9.73020895656121E-17,1.33924836902177E-16,
-1.));
#124386=DIRECTION('ref_axis',(0.,1.,1.12832121675104E-16));
#124387=DIRECTION('center_axis',(0.951131423661011,-0.308786358061005,0.));
#124388=DIRECTION('ref_axis',(0.308786358061005,0.95113142366101,0.));
#124389=DIRECTION('center_axis',(0.16375573087775,0.503988317040599,-0.848044713969304));
#124390=DIRECTION('ref_axis',(-3.99459261142949E-15,0.859649189130456,0.510884792910642));
#124391=DIRECTION('center_axis',(0.163755570286399,0.503987822791167,0.848045038708674));
#124392=DIRECTION('ref_axis',(4.51011726205046E-15,-0.859649495083727,0.510884278092695));
#124393=DIRECTION('center_axis',(0.163755716974444,0.503988355850892,-0.848044693589259));
#124394=DIRECTION('ref_axis',(-0.266368911007828,-0.80512929187988,-0.529919264233247));
#124395=DIRECTION('center_axis',(0.163755751065492,0.503988379171991,-0.848044673146743));
#124396=DIRECTION('ref_axis',(-3.74794587153715E-15,0.859649150669473,0.510884857627679));
#124397=DIRECTION('center_axis',(-0.163755599580069,-0.50398784273681,-0.848045021198562));
#124398=DIRECTION('ref_axis',(0.257959309136819,0.807862963765655,-0.529919264233172));
#124399=DIRECTION('center_axis',(0.1637555876299,0.503987876168973,0.848045003637587));
#124400=DIRECTION('ref_axis',(1.15652631111913E-15,-0.859649462041495,0.510884333691853));
#124401=DIRECTION('center_axis',(0.95097670255072,-0.309262527968972,0.));
#124402=DIRECTION('ref_axis',(0.309262527968972,0.95097670255072,0.));
#124403=DIRECTION('center_axis',(0.309016994374964,0.951056516295148,8.44187456091391E-15));
#124404=DIRECTION('ref_axis',(-0.951056516295148,0.309016994374964,-7.18667850250016E-29));
#124405=DIRECTION('center_axis',(-9.73020895656121E-17,1.33924836902177E-16,
-1.));
#124406=DIRECTION('ref_axis',(0.,1.,1.20114286872534E-16));
#124407=DIRECTION('center_axis',(0.951136266645023,-0.308771440182812,9.1132642300708E-15));
#124408=DIRECTION('ref_axis',(0.308771440182812,0.951136266645023,7.06407243348961E-29));
#124409=DIRECTION('center_axis',(0.309016994374957,0.95105651629515,-4.35148173242984E-17));
#124410=DIRECTION('ref_axis',(-0.95105651629515,0.309016994374957,4.68049650745012E-31));
#124411=DIRECTION('center_axis',(0.267642920194536,0.823622990674872,-0.500012436346858));
#124412=DIRECTION('ref_axis',(0.153571010754701,0.475845712129453,0.866017784403873));
#124413=DIRECTION('center_axis',(-0.163755751065471,-0.503988379172015,
0.848044673146733));
#124414=DIRECTION('ref_axis',(-4.07962663151818E-15,-0.859649150669459,
-0.510884857627703));
#124415=DIRECTION('center_axis',(-0.154510035624795,-0.475533025683541,
0.866022511471545));
#124416=DIRECTION('ref_axis',(-0.263355672637406,-0.825011387612138,-0.499999999999994));
#124417=DIRECTION('center_axis',(0.154510049384271,0.475533035318079,-0.866022503726344));
#124418=DIRECTION('ref_axis',(-3.78698134078517E-16,0.87654878801247,0.481313018974005));
#124419=DIRECTION('center_axis',(-0.163755716848899,-0.503988355687507,
0.8480446937106));
#124420=DIRECTION('ref_axis',(-0.257746148182604,-0.807930997357781,-0.529919264233234));
#124421=DIRECTION('center_axis',(-0.163755730877757,-0.503988317040559,
0.848044713969326));
#124422=DIRECTION('ref_axis',(-3.38818205240043E-15,-0.859649189130478,
-0.510884792910604));
#124423=DIRECTION('center_axis',(0.309016994374964,0.951056516295148,0.));
#124424=DIRECTION('ref_axis',(-0.951056516295148,0.309016994374964,0.));
#124425=DIRECTION('center_axis',(-0.309016994374964,-0.951056516295148,
0.));
#124426=DIRECTION('ref_axis',(0.951056516295148,-0.309016994374964,0.));
#124427=DIRECTION('center_axis',(0.309016994374957,0.95105651629515,-4.35148173242984E-17));
#124428=DIRECTION('ref_axis',(-0.95105651629515,0.309016994374957,4.68049650745012E-31));
#124429=DIRECTION('center_axis',(0.309016994374964,0.951056516295148,1.68837491218278E-14));
#124430=DIRECTION('ref_axis',(-0.951056516295148,0.309016994374964,-1.43733570050003E-28));
#124431=DIRECTION('center_axis',(0.309016994374957,0.95105651629515,-4.35148173242984E-17));
#124432=DIRECTION('ref_axis',(-0.95105651629515,0.309016994374957,4.68049650745012E-31));
#124433=DIRECTION('center_axis',(-0.26765302593251,-0.823639804208764,-0.499979330204879));
#124434=DIRECTION('ref_axis',(0.155418826437838,0.475210466541855,-0.86603695121961));
#124435=DIRECTION('center_axis',(0.154510091261982,0.47553316420442,0.866022425483281));
#124436=DIRECTION('ref_axis',(4.67804569173509E-15,-0.876548714628831,0.481313152617445));
#124437=DIRECTION('center_axis',(0.154510094034566,0.475533172737486,0.866022420303106));
#124438=DIRECTION('ref_axis',(0.951056516295455,-0.309016994374019,-5.94450122008058E-13));
#124439=DIRECTION('center_axis',(-0.203370361063959,-0.456777309671768,
0.866022508720031));
#124440=DIRECTION('ref_axis',(-0.913545457642825,0.406736643075296,-3.49676543997941E-13));
#124441=DIRECTION('center_axis',(-0.352213899943218,-0.791159233140749,
0.500012436348268));
#124442=DIRECTION('ref_axis',(-0.20427742790161,-0.456381342242989,-0.866017784403063));
#124443=DIRECTION('center_axis',(0.203370364581912,0.456777317573273,-0.86602250372631));
#124444=DIRECTION('ref_axis',(5.88898682911472E-15,0.884507036382098,0.466526850878444));
#124445=DIRECTION('center_axis',(0.406736643075807,0.913545457642598,0.));
#124446=DIRECTION('ref_axis',(-0.913545457642598,0.406736643075807,0.));
#124447=DIRECTION('center_axis',(-0.40673664307581,-0.913545457642596,5.72753959967211E-17));
#124448=DIRECTION('ref_axis',(0.913545457642596,-0.40673664307581,-6.16988091840288E-33));
#124449=DIRECTION('center_axis',(-0.406736643075807,-0.913545457642598,
0.));
#124450=DIRECTION('ref_axis',(0.913545457642598,-0.406736643075807,0.));
#124451=DIRECTION('center_axis',(-0.40673664307581,-0.913545457642596,5.72753959967211E-17));
#124452=DIRECTION('ref_axis',(0.913545457642596,-0.40673664307581,-6.16988091840288E-33));
#124453=DIRECTION('center_axis',(0.406736643075817,0.913545457642594,0.));
#124454=DIRECTION('ref_axis',(-0.913545457642593,0.406736643075817,0.));
#124455=DIRECTION('center_axis',(-0.215539595588313,-0.484109857923785,
-0.848045003637566));
#124456=DIRECTION('ref_axis',(-3.45358436037744E-15,0.868458021515986,-0.495762710240029));
#124457=DIRECTION('center_axis',(0.20337041970248,0.456777441376083,0.866022425483287));
#124458=DIRECTION('ref_axis',(-1.65090401241273E-16,-0.884506966812053,
0.46652698277907));
#124459=DIRECTION('center_axis',(0.215539603856733,0.48410982330642,0.848045021297519));
#124460=DIRECTION('ref_axis',(0.34886470904002,0.772967650151669,-0.529919264233175));
#124461=DIRECTION('center_axis',(-0.21553957276031,-0.484109806651251,-0.848045038708671));
#124462=DIRECTION('ref_axis',(-1.58448265001912E-15,0.86845805294998,-0.495762655175165));
#124463=DIRECTION('center_axis',(0.20337043494579,0.456777449752126,0.866022417485774));
#124464=DIRECTION('ref_axis',(0.356394722167848,0.789292595943303,-0.499999999999984));
#124465=DIRECTION('center_axis',(0.352217640366796,0.79117849009036,0.499979330205544));
#124466=DIRECTION('ref_axis',(-0.202479170978949,-0.457145692796707,0.866036951219228));
#124467=DIRECTION('center_axis',(0.913446798847318,-0.406958162070241,-2.49539780475005E-14));
#124468=DIRECTION('ref_axis',(0.406958162070241,0.913446798847317,-4.8143736717754E-28));
#124469=DIRECTION('center_axis',(-0.40673664307581,-0.913545457642596,5.72753959967211E-17));
#124470=DIRECTION('ref_axis',(0.913545457642596,-0.40673664307581,-6.16988091840288E-33));
#124471=DIRECTION('center_axis',(0.406736643075817,0.913545457642594,0.));
#124472=DIRECTION('ref_axis',(-0.913545457642593,0.406736643075817,0.));
#124473=DIRECTION('center_axis',(-8.35415108931894E-17,1.28642645648558E-16,
-1.));
#124474=DIRECTION('ref_axis',(0.,1.,1.12832121675104E-16));
#124475=DIRECTION('center_axis',(0.913644062717548,-0.406515100163541,0.));
#124476=DIRECTION('ref_axis',(0.406515100163541,0.913644062717548,0.));
#124477=DIRECTION('center_axis',(0.215539784135082,0.484110281406712,-0.848044713969326));
#124478=DIRECTION('ref_axis',(3.15501118393508E-15,0.868457761888289,0.495763165045553));
#124479=DIRECTION('center_axis',(0.215539572760321,0.484109806651275,0.848045038708655));
#124480=DIRECTION('ref_axis',(-2.32320804316489E-15,-0.868458052949965,
0.495762655175191));
#124481=DIRECTION('center_axis',(0.215539774369014,0.48411032145577,-0.848044693589286));
#124482=DIRECTION('ref_axis',(-0.349068641855651,-0.772875576446536,-0.529919264233229));
#124483=DIRECTION('center_axis',(0.215539810706709,0.484110341087599,-0.848044673146742));
#124484=DIRECTION('ref_axis',(-3.47902836708183E-15,0.868457725299276,0.495763229140693));
#124485=DIRECTION('center_axis',(-0.215539603978092,-0.484109823425721,
-0.848045021198571));
#124486=DIRECTION('ref_axis',(0.340990855174584,0.77647331575649,-0.529919264233173));
#124487=DIRECTION('center_axis',(0.215539595588318,0.484109857923797,0.848045003637558));
#124488=DIRECTION('ref_axis',(6.38857881715217E-15,-0.86845802151598,0.49576271024004));
#124489=DIRECTION('center_axis',(0.913440415876953,-0.406972488803039,-2.71806413419043E-15));
#124490=DIRECTION('ref_axis',(0.406972488803039,0.913440415876953,-4.73617210527067E-29));
#124491=DIRECTION('center_axis',(0.406736643075807,0.913545457642598,1.11114268233636E-14));
#124492=DIRECTION('ref_axis',(-0.913545457642598,0.406736643075807,1.88066567154315E-32));
#124493=DIRECTION('center_axis',(-8.35415108931894E-17,1.28642645648558E-16,
-1.));
#124494=DIRECTION('ref_axis',(0.,1.,1.20114286872534E-16));
#124495=DIRECTION('center_axis',(0.913650438514062,-0.40650077023674,0.));
#124496=DIRECTION('ref_axis',(0.40650077023674,0.913650438514061,0.));
#124497=DIRECTION('center_axis',(0.40673664307581,0.913545457642596,-5.72753959967211E-17));
#124498=DIRECTION('ref_axis',(-0.913545457642596,0.40673664307581,8.86064060326668E-32));
#124499=DIRECTION('center_axis',(0.352268789801539,0.791134794600438,-0.500012436349619));
#124500=DIRECTION('ref_axis',(0.202469153665814,0.457186437805111,0.866017784402215));
#124501=DIRECTION('center_axis',(-0.215539810706676,-0.484110341087619,
0.848044673146739));
#124502=DIRECTION('ref_axis',(-2.55985226452489E-15,-0.868457725299266,
-0.49576322914071));
#124503=DIRECTION('center_axis',(-0.203370349888124,-0.456777309430842,
0.866022511471557));
#124504=DIRECTION('ref_axis',(-0.348150155229772,-0.792963725156138,-0.499999999999987));
#124505=DIRECTION('center_axis',(0.203370364581896,0.456777317573237,-0.866022503726332));
#124506=DIRECTION('ref_axis',(-3.435979432868E-16,0.884507036382118,0.466526850878406));
#124507=DIRECTION('center_axis',(-0.215539774216652,-0.48411032131109,0.848044693710602));
#124508=DIRECTION('ref_axis',(-0.340785973383132,-0.776563258041383,-0.529919264233207));
#124509=DIRECTION('center_axis',(-0.215539784135111,-0.484110281406697,
0.848044713969328));
#124510=DIRECTION('ref_axis',(-4.1843617536873E-16,-0.868457761888296,-0.49576316504554));
#124511=DIRECTION('center_axis',(0.406736643075807,0.913545457642598,0.));
#124512=DIRECTION('ref_axis',(-0.913545457642598,0.406736643075807,0.));
#124513=DIRECTION('center_axis',(-0.406736643075817,-0.913545457642594,
0.));
#124514=DIRECTION('ref_axis',(0.913545457642593,-0.406736643075817,0.));
#124515=DIRECTION('center_axis',(0.40673664307581,0.913545457642596,-5.72753959967211E-17));
#124516=DIRECTION('ref_axis',(-0.913545457642596,0.40673664307581,8.86064060326668E-32));
#124517=DIRECTION('center_axis',(0.406736643075807,0.913545457642598,-1.11114268233636E-14));
#124518=DIRECTION('ref_axis',(-0.913545457642598,0.406736643075807,-1.88066567154315E-32));
#124519=DIRECTION('center_axis',(0.40673664307581,0.913545457642596,-5.72753959967211E-17));
#124520=DIRECTION('ref_axis',(-0.913545457642596,0.40673664307581,8.86064060326668E-32));
#124521=DIRECTION('center_axis',(-0.352280597670949,-0.791150459692801,
-0.499979330205227));
#124522=DIRECTION('ref_axis',(0.204240445640436,0.456361522794359,-0.86603695121941));
#124523=DIRECTION('center_axis',(0.203370419702468,0.456777441376069,0.866022425483298));
#124524=DIRECTION('ref_axis',(6.03968553444511E-15,-0.884506966812061,0.466526982779053));
#124525=DIRECTION('center_axis',(0.203370423353836,0.456777449577125,0.866022420300248));
#124526=DIRECTION('ref_axis',(0.91354545764332,-0.406736643074185,-1.04902962708698E-12));
#124527=DIRECTION('center_axis',(-0.250002507181426,-0.433017044457782,
0.866022508721366));
#124528=DIRECTION('ref_axis',(-0.866025403785938,0.499999999997404,-1.74838271999619E-12));
#124529=DIRECTION('center_axis',(-0.43298309418575,-0.750008802379122,0.500012436348507));
#124530=DIRECTION('ref_axis',(-0.250863215204664,-0.432528431845965,-0.866017784402866));
#124531=DIRECTION('center_axis',(0.250002511507219,0.433017051950267,-0.866022503726308));
#124532=DIRECTION('ref_axis',(2.04174131109056E-15,0.894424794863788,0.447218387740118));
#124533=DIRECTION('center_axis',(0.499999999999998,0.86602540378444,0.));
#124534=DIRECTION('ref_axis',(-0.86602540378444,0.499999999999998,0.));
#124535=DIRECTION('center_axis',(-0.50000000000001,-0.866025403784433,7.04084534449567E-17));
#124536=DIRECTION('ref_axis',(0.866025403784433,-0.50000000000001,-1.10642434862234E-32));
#124537=DIRECTION('center_axis',(-0.50000000000001,-0.866025403784433,0.));
#124538=DIRECTION('ref_axis',(0.866025403784433,-0.50000000000001,0.));
#124539=DIRECTION('center_axis',(-0.50000000000001,-0.866025403784433,7.04084534449567E-17));
#124540=DIRECTION('ref_axis',(0.866025403784433,-0.50000000000001,-1.10642434862234E-32));
#124541=DIRECTION('center_axis',(0.499999999999998,0.86602540378444,0.));
#124542=DIRECTION('ref_axis',(-0.86602540378444,0.499999999999998,0.));
#124543=DIRECTION('center_axis',(-0.264962106632877,-0.458927830768628,
-0.848045003637584));
#124544=DIRECTION('ref_axis',(-3.91597869182367E-15,0.879478602053331,-0.475938429348081));
#124545=DIRECTION('center_axis',(0.250002579266714,0.433017169313217,0.866022425483289));
#124546=DIRECTION('ref_axis',(4.16344728135109E-15,-0.894424730216417,0.447218517033106));
#124547=DIRECTION('center_axis',(0.264962111231692,0.458927795480013,0.848045021297513));
#124548=DIRECTION('ref_axis',(0.427750712286238,0.732266960563717,-0.52991926423314));
#124549=DIRECTION('center_axis',(-0.264962078570518,-0.458927782163196,
-0.848045038708653));
#124550=DIRECTION('ref_axis',(3.68379810748961E-15,0.879478631391255,-0.475938375135022));
#124551=DIRECTION('center_axis',(0.250002595294356,0.433017176054468,0.866022417485772));
#124552=DIRECTION('ref_axis',(0.436945896706248,0.747715375896206,-0.499999999999968));
#124553=DIRECTION('center_axis',(0.432988827019129,0.750027562856271,0.499979330205241));
#124554=DIRECTION('ref_axis',(-0.249154705657373,-0.433476564270065,0.866036951219408));
#124555=DIRECTION('center_axis',(0.865904130412325,-0.500209992837883,0.));
#124556=DIRECTION('ref_axis',(0.500209992837883,0.865904130412325,0.));
#124557=DIRECTION('center_axis',(-0.50000000000001,-0.866025403784433,7.04084534449567E-17));
#124558=DIRECTION('ref_axis',(0.866025403784433,-0.50000000000001,-1.10642434862234E-32));
#124559=DIRECTION('center_axis',(0.50000000000001,0.866025403784433,0.));
#124560=DIRECTION('ref_axis',(-0.866025403784433,0.50000000000001,0.));
#124561=DIRECTION('center_axis',(-7.04084534449538E-17,1.2195101864901E-16,
-1.));
#124562=DIRECTION('ref_axis',(0.,1.,1.12832121675104E-16));
#124563=DIRECTION('center_axis',(0.866146626230604,-0.499789977760002,0.));
#124564=DIRECTION('ref_axis',(0.499789977760002,0.866146626230603,0.));
#124565=DIRECTION('center_axis',(0.264962338412816,0.458928232223194,-0.84804471396932));
#124566=DIRECTION('ref_axis',(3.75627101917228E-15,0.879478359737748,0.475938877118692));
#124567=DIRECTION('center_axis',(0.264962078570517,0.45892778216318,0.848045038708662));
#124568=DIRECTION('ref_axis',(3.56607010359993E-15,-0.879478631391266,0.475938375135003));
#124569=DIRECTION('center_axis',(0.264962332885149,0.458928273074468,-0.848044693589286));
#124570=DIRECTION('ref_axis',(-0.427943903622742,-0.732154074458846,-0.529919264233185));
#124571=DIRECTION('center_axis',(0.264962371077225,0.458928288799661,-0.848044673146733));
#124572=DIRECTION('ref_axis',(2.91201203045915E-15,0.879478325588505,0.475938940222419));
#124573=DIRECTION('center_axis',(-0.264962111366864,-0.458927795584814,
-0.848045021198567));
#124574=DIRECTION('ref_axis',(0.42028643407695,0.736576463597214,-0.529919264233245));
#124575=DIRECTION('center_axis',(0.264962106632849,0.458927830768566,0.848045003637626));
#124576=DIRECTION('ref_axis',(3.02991594379835E-15,-0.879478602053368,0.475938429348013));
#124577=DIRECTION('center_axis',(0.86589628485713,-0.500223573885338,2.36549702850838E-14));
#124578=DIRECTION('ref_axis',(0.500223573885338,0.86589628485713,2.17961681937253E-28));
#124579=DIRECTION('center_axis',(0.50000000000001,0.866025403784433,0.));
#124580=DIRECTION('ref_axis',(-0.866025403784433,0.50000000000001,0.));
#124581=DIRECTION('center_axis',(-7.04084534449538E-17,1.2195101864901E-16,
-1.));
#124582=DIRECTION('ref_axis',(0.,1.,1.20114286872534E-16));
#124583=DIRECTION('center_axis',(0.866154464985094,-0.499776392786199,0.));
#124584=DIRECTION('ref_axis',(0.499776392786199,0.866154464985094,0.));
#124585=DIRECTION('center_axis',(0.50000000000001,0.866025403784433,-7.04084534449567E-17));
#124586=DIRECTION('ref_axis',(-0.866025403784433,0.50000000000001,-2.26108826570355E-32));
#124587=DIRECTION('center_axis',(0.433035128829351,0.749978760163112,-0.500012436349286));
#124588=DIRECTION('ref_axis',(0.249149002230563,0.433518133168907,0.866017784402411));
#124589=DIRECTION('center_axis',(-0.264962371077261,-0.458928288799629,
0.848044673146739));
#124590=DIRECTION('ref_axis',(1.3237123733169E-15,-0.879478325588521,-0.475938940222391));
#124591=DIRECTION('center_axis',(-0.250002496042324,-0.433017045388671,
0.86602251147154));
#124592=DIRECTION('ref_axis',(-0.429130231858343,-0.752228186194332,-0.49999999999999));
#124593=DIRECTION('center_axis',(0.250002511507148,0.433017051950192,-0.866022503726366));
#124594=DIRECTION('ref_axis',(-4.43899159512102E-15,0.894424794863831,0.447218387740031));
#124595=DIRECTION('center_axis',(-0.26496233272356,-0.458928272943599,0.848044693710594));
#124596=DIRECTION('ref_axis',(-0.420092076171116,-0.73668732915174,-0.529919264233257));
#124597=DIRECTION('center_axis',(-0.264962338412833,-0.458928232223181,
0.848044713969322));
#124598=DIRECTION('ref_axis',(5.09612267090991E-15,-0.879478359737755,-0.475938877118678));
#124599=DIRECTION('center_axis',(0.50000000000001,0.866025403784433,1.36592399683221E-14));
#124600=DIRECTION('ref_axis',(-0.866025403784433,0.50000000000001,1.17750412048402E-31));
#124601=DIRECTION('center_axis',(-0.500000000000034,-0.866025403784419,
0.));
#124602=DIRECTION('ref_axis',(0.866025403784419,-0.500000000000034,0.));
#124603=DIRECTION('center_axis',(0.50000000000001,0.866025403784433,-7.04084534449567E-17));
#124604=DIRECTION('ref_axis',(-0.866025403784433,0.50000000000001,-2.26108826570355E-32));
#124605=DIRECTION('center_axis',(0.50000000000001,0.866025403784433,3.36577552674936E-14));
#124606=DIRECTION('ref_axis',(-0.866025403784433,0.50000000000001,4.78353594691771E-31));
#124607=DIRECTION('center_axis',(0.50000000000001,0.866025403784433,-7.04084534449567E-17));
#124608=DIRECTION('ref_axis',(-0.866025403784433,0.50000000000001,-2.26108826570355E-32));
#124609=DIRECTION('center_axis',(-0.433048509462144,-0.74999310518159,-0.499979330205452));
#124610=DIRECTION('ref_axis',(0.250824363787036,0.432512586699685,-0.866036951219275));
#124611=DIRECTION('center_axis',(0.250002579266705,0.433017169313187,0.866022425483307));
#124612=DIRECTION('ref_axis',(-4.67813616211968E-15,-0.894424730216432,
0.447218517033075));
#124613=DIRECTION('center_axis',(0.250002583754379,0.433017177086056,0.866022420301321));
#124614=DIRECTION('ref_axis',(0.866025403784735,-0.499999999999487,-3.84644196594952E-13));
#124615=DIRECTION('center_axis',(-0.293895573516442,-0.404512553894514,
0.86602250871971));
#124616=DIRECTION('ref_axis',(-0.809016994376793,0.587785252289932,-1.81831802877876E-12));
#124617=DIRECTION('center_axis',(-0.509008435041602,-0.700641118228716,
0.500012436349051));
#124618=DIRECTION('ref_axis',(-0.294700492590666,-0.403936649445632,-0.866017784402523));
#124619=DIRECTION('center_axis',(0.293895578599988,0.40451256089148,-0.866022503726315));
#124620=DIRECTION('ref_axis',(4.72353162256085E-15,0.906035256115477,0.423202214875775));
#124621=DIRECTION('center_axis',(0.587785252292496,0.809016994374931,0.));
#124622=DIRECTION('ref_axis',(-0.809016994374931,0.587785252292496,0.));
#124623=DIRECTION('center_axis',(-0.587785252292482,-0.809016994374941,
8.2770101143333E-17));
#124624=DIRECTION('ref_axis',(0.809016994374941,-0.587785252292482,1.04582204444099E-33));
#124625=DIRECTION('center_axis',(-0.587785252292496,-0.809016994374931,
-3.21147992436152E-14));
#124626=DIRECTION('ref_axis',(0.809016994374931,-0.587785252292496,2.30136499084345E-30));
#124627=DIRECTION('center_axis',(-0.587785252292482,-0.809016994374941,
8.2770101143333E-17));
#124628=DIRECTION('ref_axis',(0.809016994374941,-0.587785252292482,1.04582204444099E-33));
#124629=DIRECTION('center_axis',(0.58778525229247,0.80901699437495,0.));
#124630=DIRECTION('ref_axis',(-0.80901699437495,0.58778525229247,0.));
#124631=DIRECTION('center_axis',(-0.31148163739031,-0.428717694262756,-0.848045003637588));
#124632=DIRECTION('ref_axis',(-6.37487263847381E-15,0.892442058026274,-0.451162025292277));
#124633=DIRECTION('center_axis',(0.293895658256118,0.404512670528671,0.866022425483293));
#124634=DIRECTION('ref_axis',(1.8194066783722E-15,-0.906035197473499,0.423202340422589));
#124635=DIRECTION('center_axis',(0.311481638274036,0.428717658687681,0.848045021297499));
#124636=DIRECTION('ref_axis',(0.50195018920892,0.683543400924673,-0.529919264233204));
#124637=DIRECTION('center_axis',(-0.311481604401037,-0.428717648856917,
-0.848045038708649));
#124638=DIRECTION('ref_axis',(7.95334372440912E-15,0.892442084777736,-0.451161972375297));
#124639=DIRECTION('center_axis',(0.293895674898826,0.404512675558928,0.866022417485784));
#124640=DIRECTION('ref_axis',(0.51270980056614,0.697946029721123,-0.49999999999995));
#124641=DIRECTION('center_axis',(0.509016097474113,0.700659176689997,0.499979330205079));
#124642=DIRECTION('ref_axis',(-0.293100449236466,-0.405058175796775,0.866036951219503));
#124643=DIRECTION('center_axis',(0.808874435122379,-0.587981418248444,0.));
#124644=DIRECTION('ref_axis',(0.587981418248444,0.808874435122379,0.));
#124645=DIRECTION('center_axis',(-0.587785252292482,-0.809016994374941,
8.2770101143333E-17));
#124646=DIRECTION('ref_axis',(0.809016994374941,-0.587785252292482,1.04582204444099E-33));
#124647=DIRECTION('center_axis',(0.58778525229247,0.80901699437495,0.));
#124648=DIRECTION('ref_axis',(-0.80901699437495,0.58778525229247,0.));
#124649=DIRECTION('center_axis',(-5.80468057465775E-17,1.13923270769251E-16,
-1.));
#124650=DIRECTION('ref_axis',(0.,1.,1.12832121675104E-16));
#124651=DIRECTION('center_axis',(0.809159506053906,-0.587589051772239,0.));
#124652=DIRECTION('ref_axis',(0.587589051772239,0.809159506053906,0.));
#124653=DIRECTION('center_axis',(0.3114819098639,0.428718069290558,-0.848044713969325));
#124654=DIRECTION('ref_axis',(1.92114153099776E-15,0.892441837073387,0.451162462358159));
#124655=DIRECTION('center_axis',(0.311481604401026,0.428717648856902,0.84804503870866));
#124656=DIRECTION('ref_axis',(6.88023766601185E-16,-0.892442084777746,0.451161972375277));
#124657=DIRECTION('center_axis',(0.311481908636186,0.428718110496172,-0.848044693589289));
#124658=DIRECTION('ref_axis',(-0.502130522426461,-0.683410939217635,-0.529919264233147));
#124659=DIRECTION('center_axis',(0.311481948263223,0.428718122142731,-0.848044673146738));
#124660=DIRECTION('ref_axis',(1.34798612095186E-15,0.892441805934764,0.451162523953283));
#124661=DIRECTION('center_axis',(-0.311481638423146,-0.428717658775068,
-0.848045021198555));
#124662=DIRECTION('ref_axis',(0.494977266815938,0.688609525587588,-0.529919264233205));
#124663=DIRECTION('center_axis',(0.311481637390356,0.428717694262819,0.84804500363754));
#124664=DIRECTION('ref_axis',(-5.56364179183466E-15,-0.892442058026235,
0.451162025292353));
#124665=DIRECTION('center_axis',(0.808865212939996,-0.58799410481359,-3.21262103104279E-14));
#124666=DIRECTION('ref_axis',(0.58799410481359,0.808865212939996,4.78933061976136E-28));
#124667=DIRECTION('center_axis',(0.587785252292496,0.809016994374931,-3.21147992436152E-14));
#124668=DIRECTION('ref_axis',(-0.809016994374931,0.587785252292496,2.30136499084345E-30));
#124669=DIRECTION('center_axis',(-5.80468057465775E-17,1.13923270769251E-16,
-1.));
#124670=DIRECTION('ref_axis',(0.,1.,1.20114286872534E-16));
#124671=DIRECTION('center_axis',(0.80916872188328,-0.587576360591353,-3.21033860361202E-14));
#124672=DIRECTION('ref_axis',(0.587576360591353,0.80916872188328,4.80261672572901E-28));
#124673=DIRECTION('center_axis',(0.587785252292482,0.809016994374941,-8.2770101143333E-17));
#124674=DIRECTION('ref_axis',(-0.809016994374941,0.587785252292482,4.73588184773858E-32));
#124675=DIRECTION('center_axis',(0.509057044368194,0.700605801485152,-0.500012436349803));
#124676=DIRECTION('ref_axis',(0.293099122184562,0.405100113149701,0.86601778440211));
#124677=DIRECTION('center_axis',(-0.311481948263288,-0.428718122142702,
0.848044673146728));
#124678=DIRECTION('ref_axis',(6.50740225724504E-15,-0.892441805934775,-0.451162523953261));
#124679=DIRECTION('center_axis',(-0.293895562534375,-0.40451255598208,0.866022511471525));
#124680=DIRECTION('ref_axis',(-0.505408667883912,-0.70325107780065,-0.500000000000034));
#124681=DIRECTION('center_axis',(0.293895578599968,0.404512560891387,-0.866022503726365));
#124682=DIRECTION('ref_axis',(1.55256022332075E-15,0.906035256115524,0.423202214875674));
#124683=DIRECTION('center_axis',(-0.311481908459053,-0.42871811038485,0.848044693710626));
#124684=DIRECTION('ref_axis',(-0.494795562234247,-0.688740099738556,-0.529919264233166));
#124685=DIRECTION('center_axis',(-0.311481909863969,-0.428718069290495,
0.848044713969331));
#124686=DIRECTION('ref_axis',(1.5898874044363E-15,-0.892441837073416,-0.451162462358103));
#124687=DIRECTION('center_axis',(0.587785252292496,0.809016994374931,0.));
#124688=DIRECTION('ref_axis',(-0.809016994374931,0.587785252292496,0.));
#124689=DIRECTION('center_axis',(-0.587785252292496,-0.809016994374931,
0.));
#124690=DIRECTION('ref_axis',(0.809016994374931,-0.587785252292496,0.));
#124691=DIRECTION('center_axis',(0.587785252292482,0.809016994374941,-8.2770101143333E-17));
#124692=DIRECTION('ref_axis',(-0.809016994374941,0.587785252292482,4.73588184773858E-32));
#124693=DIRECTION('center_axis',(0.587785252292496,0.809016994374931,-4.42022290584682E-14));
#124694=DIRECTION('ref_axis',(-0.809016994374931,0.587785252292496,1.69177565650547E-30));
#124695=DIRECTION('center_axis',(0.587785252292482,0.809016994374941,-8.2770101143333E-17));
#124696=DIRECTION('ref_axis',(-0.809016994374941,0.587785252292482,4.73588184773858E-32));
#124697=DIRECTION('center_axis',(-0.50907185116306,-0.700618669263837,-0.499979330205146));
#124698=DIRECTION('ref_axis',(0.294660197696144,0.403924952207911,-0.866036951219465));
#124699=DIRECTION('center_axis',(0.293895658256114,0.404512670528666,0.866022425483297));
#124700=DIRECTION('ref_axis',(-6.85542257558146E-17,-0.906035197473502,
0.423202340422583));
#124701=DIRECTION('center_axis',(0.293895663530901,0.404512677788762,0.866022420302094));
#124702=DIRECTION('ref_axis',(0.809016994373366,-0.58778525229465,1.53857678639347E-12));
#124703=DIRECTION('center_axis',(-0.334568658443799,-0.371576139137306,
0.866022508720721));
#124704=DIRECTION('ref_axis',(-0.743144825476915,0.66913060635939,4.19611852791889E-13));
#124705=DIRECTION('center_axis',(-0.579456972966298,-0.643597063368579,
0.500012436349413));
#124706=DIRECTION('ref_axis',(-0.335308969655448,-0.370919252624417,-0.866017784402345));
#124707=DIRECTION('center_axis',(0.334568664232119,0.37157614556582,-0.866022503726309));
#124708=DIRECTION('ref_axis',(2.56241420419672E-15,0.918982183096524,0.394299058014532));
#124709=DIRECTION('center_axis',(0.669130606358875,0.743144825477379,0.));
#124710=DIRECTION('ref_axis',(-0.743144825477379,0.669130606358875,0.));
#124711=DIRECTION('center_axis',(-0.669130606358867,-0.743144825477386,
9.42249022928259E-17));
#124712=DIRECTION('ref_axis',(0.743144825477386,-0.669130606358867,1.14423954767457E-32));
#124713=DIRECTION('center_axis',(-0.669130606358845,-0.743144825477406,
4.06031740096479E-14));
#124714=DIRECTION('ref_axis',(0.743144825477406,-0.669130606358845,-1.17388982313054E-30));
#124715=DIRECTION('center_axis',(-0.669130606358867,-0.743144825477386,
9.42249022928259E-17));
#124716=DIRECTION('ref_axis',(0.743144825477386,-0.669130606358867,-3.88054752867469E-33));
#124717=DIRECTION('center_axis',(0.669130606358845,0.743144825477406,0.));
#124718=DIRECTION('ref_axis',(-0.743144825477406,0.669130606358845,0.));
#124719=DIRECTION('center_axis',(-0.354588510146749,-0.393810436983632,
-0.848045003637584));
#124720=DIRECTION('ref_axis',(-5.89688827602511E-16,0.906978223357768,-0.421177518814558));
#124721=DIRECTION('center_axis',(0.334568754912034,0.371576246276112,0.866022425483293));
#124722=DIRECTION('ref_axis',(2.56170689995423E-15,-0.918982131463647,0.394299178353863));
#124723=DIRECTION('center_axis',(0.354588507310876,0.39381040150757,0.848045021297508));
#124724=DIRECTION('ref_axis',(0.570650194839117,0.627330796729033,-0.529919264233142));
#124725=DIRECTION('center_axis',(-0.354588472592004,-0.393810395274862,
-0.848045038708633));
#124726=DIRECTION('ref_axis',(1.64363307278047E-15,0.906978247051285,-0.421177467792116));
#124727=DIRECTION('center_axis',(0.334568771994895,0.37157624953427,0.866022417485757));
#124728=DIRECTION('ref_axis',(0.582856348565578,0.640529840785569,-0.500000000000016));
#124729=DIRECTION('center_axis',(0.579466481046627,0.643614221961416,0.4999793302052));
#124730=DIRECTION('ref_axis',(-0.333834922962011,-0.372201885182612,0.866036951219437));
#124731=DIRECTION('center_axis',(0.742982542253377,-0.669310796197633,-7.71634144622546E-14));
#124732=DIRECTION('ref_axis',(0.669310796197633,0.742982542253377,-3.15085687395575E-28));
#124733=DIRECTION('center_axis',(-0.669130606358867,-0.743144825477386,
9.42249022928259E-17));
#124734=DIRECTION('ref_axis',(0.743144825477386,-0.669130606358867,1.14423954767457E-32));
#124735=DIRECTION('center_axis',(0.669130606358845,0.743144825477406,0.));
#124736=DIRECTION('ref_axis',(-0.743144825477406,0.669130606358845,0.));
#124737=DIRECTION('center_axis',(-4.65920045970846E-17,1.04647355694968E-16,
-1.));
#124738=DIRECTION('ref_axis',(0.,1.,1.12832121675104E-16));
#124739=DIRECTION('center_axis',(0.743307065001304,-0.668950377172438,0.));
#124740=DIRECTION('ref_axis',(0.668950377172438,0.743307065001304,0.));
#124741=DIRECTION('center_axis',(0.354588820328836,0.39381078147567,-0.848044713969332));
#124742=DIRECTION('ref_axis',(7.54048452976697E-15,0.906978027661857,0.421177940232638));
#124743=DIRECTION('center_axis',(0.354588472592016,0.393810395274875,0.848045038708621));
#124744=DIRECTION('ref_axis',(4.30002933985616E-15,-0.906978247051278,0.42117746779213));
#124745=DIRECTION('center_axis',(0.354588823409533,0.393810822588869,-0.848044693589271));
#124746=DIRECTION('ref_axis',(-0.570815694142538,-0.62718021071711,-0.52991926423316));
#124747=DIRECTION('center_axis',(0.354588864042302,0.393810830024563,-0.848044673146736));
#124748=DIRECTION('ref_axis',(-8.30756835896895E-15,0.906978000082633,0.421177999622615));
#124749=DIRECTION('center_axis',(-0.354588507465445,-0.393810401581466,
-0.848045021198564));
#124750=DIRECTION('ref_axis',(0.564245025076819,0.633098037487535,-0.529919264233234));
#124751=DIRECTION('center_axis',(0.354588510146734,0.393810436983615,0.848045003637598));
#124752=DIRECTION('ref_axis',(9.67156497587423E-15,-0.906978223357779,0.421177518814534));
#124753=DIRECTION('center_axis',(0.742972044483923,-0.669322449283885,4.02398997762811E-15));
#124754=DIRECTION('ref_axis',(0.669322449283885,0.742972044483923,8.70636259521657E-29));
#124755=DIRECTION('center_axis',(0.669130606358845,0.743144825477406,4.06031740096502E-14));
#124756=DIRECTION('ref_axis',(-0.743144825477406,0.669130606358845,-2.91235641449386E-31));
#124757=DIRECTION('center_axis',(-4.65920045970846E-17,1.04647355694968E-16,
-1.));
#124758=DIRECTION('ref_axis',(0.,1.,1.20114286872534E-16));
#124759=DIRECTION('center_axis',(0.743317556935059,-0.668938718831625,0.));
#124760=DIRECTION('ref_axis',(0.668938718831625,0.743317556935059,0.));
#124761=DIRECTION('center_axis',(0.669130606358867,0.743144825477386,-9.42249022928259E-17));
#124762=DIRECTION('ref_axis',(-0.743144825477386,0.669130606358867,8.40817423203469E-31));
#124763=DIRECTION('center_axis',(0.579501624401492,0.643556859034944,-0.500012436350447));
#124764=DIRECTION('ref_axis',(0.333837986828513,0.372243731512272,0.866017784401743));
#124765=DIRECTION('center_axis',(-0.354588864042398,-0.393810830024467,
0.848044673146741));
#124766=DIRECTION('ref_axis',(-6.88772073415207E-15,-0.906978000082671,
-0.421177999622534));
#124767=DIRECTION('center_axis',(-0.334568647742382,-0.371576142361624,
0.866022511471549));
#124768=DIRECTION('ref_axis',(-0.576149740778052,-0.646569003433809,-0.499999999999994));
#124769=DIRECTION('center_axis',(0.334568664232095,0.371576145565864,-0.866022503726299));
#124770=DIRECTION('ref_axis',(3.33579067942304E-15,0.918982183096505,0.394299058014576));
#124771=DIRECTION('center_axis',(-0.354588823227312,-0.393810822491673,
0.848044693710598));
#124772=DIRECTION('ref_axis',(-0.564077964592822,-0.633246889653118,-0.529919264233215));
#124773=DIRECTION('center_axis',(-0.354588820328848,-0.393810781475683,
0.848044713969321));
#124774=DIRECTION('ref_axis',(-1.51628995831101E-15,-0.90697802766185,-0.421177940232653));
#124775=DIRECTION('center_axis',(0.669130606358845,0.743144825477406,3.65592620896146E-14));
#124776=DIRECTION('ref_axis',(-0.743144825477406,0.669130606358845,9.99649599890217E-31));
#124777=DIRECTION('center_axis',(-0.669130606358872,-0.743144825477382,
0.));
#124778=DIRECTION('ref_axis',(0.743144825477382,-0.669130606358872,0.));
#124779=DIRECTION('center_axis',(0.669130606358867,0.743144825477386,-9.42249022928259E-17));
#124780=DIRECTION('ref_axis',(-0.743144825477386,0.669130606358867,8.40817423203469E-31));
#124781=DIRECTION('center_axis',(0.669130606358845,0.743144825477406,3.65592620896126E-14));
#124782=DIRECTION('ref_axis',(-0.743144825477406,0.669130606358845,-2.40072602627987E-31));
#124783=DIRECTION('center_axis',(0.669130606358867,0.743144825477386,-9.42249022928259E-17));
#124784=DIRECTION('ref_axis',(-0.743144825477386,0.669130606358867,8.40817423203469E-31));
#124785=DIRECTION('center_axis',(-0.579517695131705,-0.643568108591948,
-0.499979330205379));
#124786=DIRECTION('ref_axis',(0.335267672852102,0.370911831387327,-0.866036951219309));
#124787=DIRECTION('center_axis',(0.33456875491201,0.371576246276113,0.866022425483302));
#124788=DIRECTION('ref_axis',(1.51465199069959E-15,-0.918982131463649,0.394299178353861));
#124789=DIRECTION('center_axis',(0.334568760918561,0.37157625294704,0.866022420300569));
#124790=DIRECTION('ref_axis',(0.743144825473852,-0.669130606362792,3.04218591854262E-12));
#124791=DIRECTION('center_axis',(-0.371576139134505,-0.334568658441323,
0.866022508722879));
#124792=DIRECTION('ref_axis',(-0.669130606356846,0.743144825479206,1.57354444798169E-12));
#124793=DIRECTION('center_axis',(-0.643556859036478,-0.579501624401258,
0.500012436348744));
#124794=DIRECTION('ref_axis',(-0.372243731475059,-0.333837986867333,-0.866017784402775));
#124795=DIRECTION('center_axis',(0.371576145565853,0.334568664232085,-0.866022503726308));
#124796=DIRECTION('ref_axis',(-0.918982183096513,7.65889573873005E-15,-0.394299058014558));
#124797=DIRECTION('center_axis',(0.743144825477379,0.669130606358875,0.));
#124798=DIRECTION('ref_axis',(-0.669130606358875,0.743144825477379,0.));
#124799=DIRECTION('center_axis',(-0.743144825477402,-0.66913060635885,1.0464735569497E-16));
#124800=DIRECTION('ref_axis',(0.66913060635885,-0.743144825477402,-1.36521113930368E-32));
#124801=DIRECTION('center_axis',(-0.743144825477406,-0.669130606358845,
0.));
#124802=DIRECTION('ref_axis',(0.669130606358845,-0.743144825477406,0.));
#124803=DIRECTION('center_axis',(-0.743144825477402,-0.66913060635885,1.0464735569497E-16));
#124804=DIRECTION('ref_axis',(0.66913060635885,-0.743144825477402,-1.36521113930368E-32));
#124805=DIRECTION('center_axis',(0.743144825477382,0.669130606358872,0.));
#124806=DIRECTION('ref_axis',(-0.669130606358872,0.743144825477382,0.));
#124807=DIRECTION('center_axis',(-0.393810436983627,-0.354588510146745,
-0.848045003637588));
#124808=DIRECTION('ref_axis',(-0.90697822335777,-1.33133695181472E-15,0.421177518814553));
#124809=DIRECTION('center_axis',(0.371576246276117,0.334568754912014,0.866022425483298));
#124810=DIRECTION('ref_axis',(0.918982131463646,-3.28768502367003E-15,-0.394299178353865));
#124811=DIRECTION('center_axis',(0.393810430452539,0.354588475164265,0.848045021297494));
#124812=DIRECTION('ref_axis',(0.633098037499372,0.564245025063572,-0.529919264233196));
#124813=DIRECTION('center_axis',(-0.393810395274859,-0.354588472592001,
-0.848045038708636));
#124814=DIRECTION('ref_axis',(-0.906978247051286,-3.29122279906641E-15,
0.421177467792112));
#124815=DIRECTION('center_axis',(0.37157626360525,0.334568756367432,0.866022417485778));
#124816=DIRECTION('ref_axis',(0.646617000437273,0.576095872876662,-0.49999999999998));
#124817=DIRECTION('center_axis',(0.643568108591639,0.579517695132388,0.499979330204985));
#124818=DIRECTION('ref_axis',(-0.370911831408801,-0.335267672827688,0.866036951219563));
#124819=DIRECTION('center_axis',(0.668950377172403,-0.743307065001336,0.));
#124820=DIRECTION('ref_axis',(0.743307065001336,0.668950377172402,0.));
#124821=DIRECTION('center_axis',(-0.743144825477402,-0.66913060635885,1.0464735569497E-16));
#124822=DIRECTION('ref_axis',(0.66913060635885,-0.743144825477402,-1.36521113930368E-32));
#124823=DIRECTION('center_axis',(0.743144825477409,0.669130606358842,0.));
#124824=DIRECTION('ref_axis',(-0.669130606358842,0.743144825477409,0.));
#124825=DIRECTION('center_axis',(-3.61695511949404E-17,9.42249022928235E-17,
-1.));
#124826=DIRECTION('ref_axis',(0.,1.,1.12832121675104E-16));
#124827=DIRECTION('center_axis',(0.669310796197601,-0.742982542253406,0.));
#124828=DIRECTION('ref_axis',(0.742982542253406,0.669310796197601,0.));
#124829=DIRECTION('center_axis',(0.393810781475729,0.354588820328856,-0.848044713969297));
#124830=DIRECTION('ref_axis',(-0.906978027661826,-7.21760554452843E-15,
-0.421177940232705));
#124831=DIRECTION('center_axis',(0.393810395274862,0.354588472592004,0.848045038708633));
#124832=DIRECTION('ref_axis',(0.906978247051285,1.62635303421704E-15,-0.421177467792116));
#124833=DIRECTION('center_axis',(0.393810788839631,0.354588860891869,-0.848044693589267));
#124834=DIRECTION('ref_axis',(-0.633246889667058,-0.564077964577223,-0.52991926423316));
#124835=DIRECTION('center_axis',(0.393810830024499,0.354588864042362,-0.848044673146741));
#124836=DIRECTION('ref_axis',(-0.906978000082659,3.44782577783986E-15,-0.421177999622559));
#124837=DIRECTION('center_axis',(-0.393810430614147,-0.354588475221364,
-0.848045021198573));
#124838=DIRECTION('ref_axis',(0.627330796753185,0.570650194812477,-0.529919264233238));
#124839=DIRECTION('center_axis',(0.39381043698369,0.354588510146801,0.848045003637535));
#124840=DIRECTION('ref_axis',(0.906978223357735,-2.65352984180235E-15,-0.421177518814628));
#124841=DIRECTION('center_axis',(0.668938718831589,-0.743317556935091,0.));
#124842=DIRECTION('ref_axis',(0.743317556935091,0.668938718831589,0.));
#124843=DIRECTION('center_axis',(0.743144825477406,0.669130606358845,0.));
#124844=DIRECTION('ref_axis',(-0.669130606358845,0.743144825477406,0.));
#124845=DIRECTION('center_axis',(-3.61695511949404E-17,9.42249022928235E-17,
-1.));
#124846=DIRECTION('ref_axis',(0.,1.,1.20114286872534E-16));
#124847=DIRECTION('center_axis',(0.669322449283883,-0.742972044483925,0.));
#124848=DIRECTION('ref_axis',(0.742972044483925,0.669322449283883,0.));
#124849=DIRECTION('center_axis',(0.743144825477402,0.66913060635885,-1.0464735569497E-16));
#124850=DIRECTION('ref_axis',(-0.66913060635885,0.743144825477402,-1.26626413714807E-30));
#124851=DIRECTION('center_axis',(0.643597063368661,0.579456972966462,-0.500012436349118));
#124852=DIRECTION('ref_axis',(0.370919252629949,0.335308969648868,0.866017784402523));
#124853=DIRECTION('center_axis',(-0.393810830024549,-0.354588864042318,
0.848044673146736));
#124854=DIRECTION('ref_axis',(0.906978000082638,-3.66139072703648E-15,0.421177999622604));
#124855=DIRECTION('center_axis',(-0.371576128832128,-0.334568662768395,
0.866022511471554));
#124856=DIRECTION('ref_axis',(-0.640578396537439,-0.582802983768563,-0.499999999999984));
#124857=DIRECTION('center_axis',(0.371576145565796,0.334568664232034,-0.866022503726352));
#124858=DIRECTION('ref_axis',(-0.91898218309654,3.67733214476396E-16,-0.394299058014493));
#124859=DIRECTION('center_axis',(-0.393810788646935,-0.354588860815713,
0.848044693710593));
#124860=DIRECTION('ref_axis',(-0.627180210735122,-0.570815694122663,-0.529919264233251));
#124861=DIRECTION('center_axis',(-0.393810781475744,-0.354588820328778,
0.848044713969322));
#124862=DIRECTION('ref_axis',(0.906978027661825,6.0864701038141E-15,0.421177940232708));
#124863=DIRECTION('center_axis',(0.743144825477406,0.669130606358845,4.0439119200333E-15));
#124864=DIRECTION('ref_axis',(-0.669130606358845,0.743144825477406,3.55234324240431E-31));
#124865=DIRECTION('center_axis',(-0.743144825477406,-0.669130606358845,
0.));
#124866=DIRECTION('ref_axis',(0.669130606358845,-0.743144825477406,0.));
#124867=DIRECTION('center_axis',(0.743144825477402,0.66913060635885,-1.0464735569497E-16));
#124868=DIRECTION('ref_axis',(-0.66913060635885,0.743144825477402,6.45362564166036E-31));
#124869=DIRECTION('center_axis',(0.743144825477406,0.669130606358845,4.04391192003308E-15));
#124870=DIRECTION('ref_axis',(-0.669130606358845,0.743144825477406,1.02141021320469E-31));
#124871=DIRECTION('center_axis',(0.743144825477402,0.66913060635885,-1.0464735569497E-16));
#124872=DIRECTION('ref_axis',(-0.66913060635885,0.743144825477402,6.45362564166036E-31));
#124873=DIRECTION('center_axis',(-0.643614221961378,-0.57946648104669,-0.499979330205176));
#124874=DIRECTION('ref_axis',(0.372201885190803,0.333834922952869,-0.866036951219441));
#124875=DIRECTION('center_axis',(0.371576246276125,0.334568754912021,0.866022425483293));
#124876=DIRECTION('ref_axis',(0.918982131463643,-6.34168247799913E-15,-0.394299178353873));
#124877=DIRECTION('center_axis',(0.371576252947737,0.334568760919143,0.866022420300046));
#124878=DIRECTION('ref_axis',(0.669130606360272,-0.743144825476121,-1.11896493554479E-12));
#124879=DIRECTION('center_axis',(-0.404512553894778,-0.29389557351658,0.866022508719539));
#124880=DIRECTION('ref_axis',(-0.587785252299528,0.809016994369821,-5.07030988789205E-12));
#124881=DIRECTION('center_axis',(-0.700605801487114,-0.509057044366917,
0.500012436348355));
#124882=DIRECTION('ref_axis',(-0.405100113158709,-0.293099122169683,-0.866017784402932));
#124883=DIRECTION('center_axis',(0.404512560891477,0.293895578600006,-0.86602250372631));
#124884=DIRECTION('ref_axis',(-0.906035256115479,9.01705582438248E-15,-0.423202214875771));
#124885=DIRECTION('center_axis',(0.80901699437495,0.58778525229247,0.));
#124886=DIRECTION('ref_axis',(-0.58778525229247,0.80901699437495,0.));
#124887=DIRECTION('center_axis',(-0.809016994374955,-0.587785252292463,
1.13923270769253E-16));
#124888=DIRECTION('ref_axis',(0.587785252292463,-0.809016994374955,7.17089999548893E-33));
#124889=DIRECTION('center_axis',(-0.80901699437495,-0.58778525229247,0.));
#124890=DIRECTION('ref_axis',(0.58778525229247,-0.80901699437495,0.));
#124891=DIRECTION('center_axis',(-0.809016994374955,-0.587785252292463,
1.13923270769253E-16));
#124892=DIRECTION('ref_axis',(0.587785252292463,-0.809016994374955,7.17089999548893E-33));
#124893=DIRECTION('center_axis',(0.80901699437495,0.58778525229247,0.));
#124894=DIRECTION('ref_axis',(-0.58778525229247,0.80901699437495,0.));
#124895=DIRECTION('center_axis',(-0.428717694262757,-0.31148163739029,-0.848045003637595));
#124896=DIRECTION('ref_axis',(-0.892442058026274,5.80484162998979E-15,0.451162025292275));
#124897=DIRECTION('center_axis',(0.404512670528679,0.293895658256096,0.866022425483297));
#124898=DIRECTION('ref_axis',(0.906035197473497,-3.36511067292208E-15,-0.423202340422593));
#124899=DIRECTION('center_axis',(0.428717684113496,0.311481603278383,0.848045021297507));
#124900=DIRECTION('ref_axis',(0.68860952557487,0.494977266833581,-0.529919264233252));
#124901=DIRECTION('center_axis',(-0.428717648856936,-0.31148160440103,-0.848045038708641));
#124902=DIRECTION('ref_axis',(-0.892442084777727,-1.51672008863495E-15,
0.451161972375314));
#124903=DIRECTION('center_axis',(0.404512687914156,0.293895657893397,0.866022417485755));
#124904=DIRECTION('ref_axis',(0.703293181141416,0.505350078025127,-0.499999999999986));
#124905=DIRECTION('center_axis',(0.700618669263901,0.509071851162835,0.499979330205284));
#124906=DIRECTION('ref_axis',(-0.403924952198554,-0.294660197709245,0.866036951219372));
#124907=DIRECTION('center_axis',(0.587589051772177,-0.809159506053951,4.42100154633563E-14));
#124908=DIRECTION('ref_axis',(0.809159506053951,0.587589051772177,1.06274147446815E-27));
#124909=DIRECTION('center_axis',(-0.809016994374955,-0.587785252292463,
1.13923270769253E-16));
#124910=DIRECTION('ref_axis',(0.587785252292463,-0.809016994374955,7.17089999548893E-33));
#124911=DIRECTION('center_axis',(0.80901699437495,0.58778525229247,0.));
#124912=DIRECTION('ref_axis',(-0.58778525229247,0.80901699437495,0.));
#124913=DIRECTION('center_axis',(-2.68936361206573E-17,8.27701011433304E-17,
-1.));
#124914=DIRECTION('ref_axis',(0.,1.,1.12832121675104E-16));
#124915=DIRECTION('center_axis',(0.587981418248456,-0.808874435122371,0.));
#124916=DIRECTION('ref_axis',(0.808874435122371,0.587981418248456,0.));
#124917=DIRECTION('center_axis',(0.428718069290566,0.311481909863963,-0.848044713969297));
#124918=DIRECTION('ref_axis',(-0.892441837073379,4.20951290950153E-15,-0.451162462358176));
#124919=DIRECTION('center_axis',(0.428717648856939,0.311481604401032,0.848045038708639));
#124920=DIRECTION('ref_axis',(0.892442084777726,6.53865308856261E-16,-0.451161972375317));
#124921=DIRECTION('center_axis',(0.428718080852843,0.311481949436789,-0.848044693589266));
#124922=DIRECTION('ref_axis',(-0.688740099740917,-0.494795562230913,-0.52991926423321));
#124923=DIRECTION('center_axis',(0.428718122142669,0.3114819482633,-0.848044673146741));
#124924=DIRECTION('ref_axis',(-0.89244180593479,-4.45144579489326E-15,-0.451162523953232));
#124925=DIRECTION('center_axis',(-0.428717684279335,-0.311481603319502,
-0.848045021198567));
#124926=DIRECTION('ref_axis',(0.683543400919167,0.501950189216426,-0.529919264233197));
#124927=DIRECTION('center_axis',(0.42871769426279,0.311481637390314,0.84804500363757));
#124928=DIRECTION('ref_axis',(0.892442058026255,-3.92099685579204E-15,-0.451162025292314));
#124929=DIRECTION('center_axis',(0.587576360591332,-0.809168721883295,1.21071329521359E-14));
#124930=DIRECTION('ref_axis',(0.809168721883294,0.587576360591332,-4.66403124080741E-29));
#124931=DIRECTION('center_axis',(0.80901699437495,0.58778525229247,-3.21147992436137E-14));
#124932=DIRECTION('ref_axis',(-0.58778525229247,0.80901699437495,6.08123400109255E-31));
#124933=DIRECTION('center_axis',(-2.68936361206573E-17,8.27701011433304E-17,
-1.));
#124934=DIRECTION('ref_axis',(0.,1.,1.20114286872534E-16));
#124935=DIRECTION('center_axis',(0.587994104813612,-0.80886521293998,-1.20677258718689E-14));
#124936=DIRECTION('ref_axis',(0.80886521293998,0.587994104813612,1.52456665748993E-28));
#124937=DIRECTION('center_axis',(0.809016994374955,0.587785252292463,-1.13923270769253E-16));
#124938=DIRECTION('ref_axis',(-0.587785252292463,0.809016994374955,-2.72904051338169E-30));
#124939=DIRECTION('center_axis',(0.700641118228982,0.509008435040225,-0.50001243635008));
#124940=DIRECTION('ref_axis',(0.403936649504382,0.294700492511635,0.866017784402014));
#124941=DIRECTION('center_axis',(-0.428718122142697,-0.311481948263293,
0.848044673146729));
#124942=DIRECTION('ref_axis',(0.892441805934777,-5.0778461836944E-15,0.451162523953257));
#124943=DIRECTION('center_axis',(-0.404512544096507,-0.293895578893441,
0.866022511471532));
#124944=DIRECTION('ref_axis',(-0.697988741332449,-0.512651652658167,-0.499999999999993));
#124945=DIRECTION('center_axis',(0.404512560891374,0.293895578599939,-0.866022503726381));
#124946=DIRECTION('ref_axis',(-0.906035256115533,6.95641201217777E-15,-0.423202214875654));
#124947=DIRECTION('center_axis',(-0.428718080655422,-0.311481949378178,
0.848044693710597));
#124948=DIRECTION('ref_axis',(-0.683410939228684,-0.50213052241134,-0.529919264233225));
#124949=DIRECTION('center_axis',(-0.428718069290593,-0.311481909863876,
0.848044713969316));
#124950=DIRECTION('ref_axis',(0.89244183707337,5.21317305093966E-15,0.451162462358194));
#124951=DIRECTION('center_axis',(0.80901699437495,0.58778525229247,-3.2114799243612E-14));
#124952=DIRECTION('ref_axis',(-0.58778525229247,0.80901699437495,-4.13565546558353E-30));
#124953=DIRECTION('center_axis',(-0.809016994374976,-0.587785252292434,
0.));
#124954=DIRECTION('ref_axis',(0.587785252292434,-0.809016994374976,0.));
#124955=DIRECTION('center_axis',(0.809016994374955,0.587785252292463,-1.13923270769253E-16));
#124956=DIRECTION('ref_axis',(-0.587785252292463,0.809016994374955,-2.72904051338169E-30));
#124957=DIRECTION('center_axis',(0.80901699437495,0.58778525229247,0.));
#124958=DIRECTION('ref_axis',(-0.58778525229247,0.80901699437495,0.));
#124959=DIRECTION('center_axis',(0.809016994374955,0.587785252292463,-1.13923270769253E-16));
#124960=DIRECTION('ref_axis',(-0.587785252292463,0.809016994374955,-2.72904051338169E-30));
#124961=DIRECTION('center_axis',(-0.700659176689738,-0.50901609747425,-0.499979330205303));
#124962=DIRECTION('ref_axis',(0.405058175803442,0.293100449227661,-0.866036951219364));
#124963=DIRECTION('center_axis',(0.404512670528659,0.293895658256089,0.866022425483309));
#124964=DIRECTION('ref_axis',(0.906035197473507,3.41535267324782E-15,-0.423202340422573));
#124965=DIRECTION('center_axis',(0.4045126777905,0.293895663532146,0.86602242030086));
#124966=DIRECTION('ref_axis',(0.587785252291003,-0.809016994376015,1.04902962708232E-12));
#124967=DIRECTION('center_axis',(-0.433017044458743,-0.250002507181973,
0.866022508720728));
#124968=DIRECTION('ref_axis',(-0.500000000003119,0.866025403782638,-2.02812395516345E-12));
#124969=DIRECTION('center_axis',(-0.749978760163342,-0.433035128829169,
0.500012436349099));
#124970=DIRECTION('ref_axis',(-0.433518133182558,-0.24914900220652,-0.866017784402495));
#124971=DIRECTION('center_axis',(0.43301705195027,0.250002511507201,-0.866022503726312));
#124972=DIRECTION('ref_axis',(-0.894424794863788,-1.72347843759609E-15,
-0.447218387740119));
#124973=DIRECTION('center_axis',(0.866025403784433,0.50000000000001,0.));
#124974=DIRECTION('ref_axis',(-0.50000000000001,0.866025403784433,0.));
#124975=DIRECTION('center_axis',(-0.866025403784445,-0.499999999999989,
1.21951018649011E-16));
#124976=DIRECTION('ref_axis',(0.499999999999989,-0.866025403784445,7.73386177718291E-33));
#124977=DIRECTION('center_axis',(-0.86602540378444,-0.499999999999998,-1.3659239968321E-14));
#124978=DIRECTION('ref_axis',(0.499999999999998,-0.86602540378444,-1.8627714006626E-28));
#124979=DIRECTION('center_axis',(-0.866025403784445,-0.499999999999989,
1.21951018649011E-16));
#124980=DIRECTION('ref_axis',(0.499999999999989,-0.866025403784445,7.73386177718291E-33));
#124981=DIRECTION('center_axis',(0.866025403784463,0.499999999999957,0.));
#124982=DIRECTION('ref_axis',(-0.499999999999957,0.866025403784463,0.));
#124983=DIRECTION('center_axis',(-0.458927830768608,-0.264962106632866,
-0.848045003637598));
#124984=DIRECTION('ref_axis',(-0.879478602053342,-2.31870210175756E-15,
0.475938429348061));
#124985=DIRECTION('center_axis',(0.43301716931321,0.250002579266718,0.866022425483292));
#124986=DIRECTION('ref_axis',(0.89442473021642,-2.13116799657304E-15,-0.447218517033099));
#124987=DIRECTION('center_axis',(0.458927817109519,0.264962073768271,0.848045021297519));
#124988=DIRECTION('ref_axis',(0.736576463609069,0.42028643405628,-0.529919264233161));
#124989=DIRECTION('center_axis',(-0.458927782163189,-0.264962078570514,
-0.848045038708658));
#124990=DIRECTION('ref_axis',(-0.879478631391259,-6.14731538978695E-15,
0.475938375135014));
#124991=DIRECTION('center_axis',(0.433017186566327,0.250002577087191,0.866022417485798));
#124992=DIRECTION('ref_axis',(0.752263934579074,0.429067561966284,-0.49999999999992));
#124993=DIRECTION('center_axis',(0.749993105181526,0.433048509462592,0.49997933020516));
#124994=DIRECTION('ref_axis',(-0.432512586703677,-0.250824363779544,0.86603695121945));
#124995=DIRECTION('center_axis',(0.499789977759954,-0.866146626230631,0.));
#124996=DIRECTION('ref_axis',(0.866146626230631,0.499789977759954,0.));
#124997=DIRECTION('center_axis',(-0.866025403784445,-0.499999999999989,
1.21951018649011E-16));
#124998=DIRECTION('ref_axis',(0.499999999999989,-0.866025403784445,7.73386177718291E-33));
#124999=DIRECTION('center_axis',(0.86602540378444,0.499999999999998,0.));
#125000=DIRECTION('ref_axis',(-0.499999999999998,0.86602540378444,0.));
#125001=DIRECTION('center_axis',(-1.88658882408992E-17,7.04084534449537E-17,
-1.));
#125002=DIRECTION('ref_axis',(0.,1.,1.12832121675104E-16));
#125003=DIRECTION('center_axis',(0.500209992837931,-0.865904130412297,0.));
#125004=DIRECTION('ref_axis',(0.865904130412297,0.500209992837931,0.));
#125005=DIRECTION('center_axis',(0.458928232223227,0.264962338412753,-0.848044713969322));
#125006=DIRECTION('ref_axis',(-0.879478359737735,3.52718193142461E-15,-0.475938877118715));
#125007=DIRECTION('center_axis',(0.458927782163212,0.264962078570527,0.848045038708642));
#125008=DIRECTION('ref_axis',(0.879478631391246,-1.38546995367359E-15,-0.475938375135038));
#125009=DIRECTION('center_axis',(0.458928247861521,0.264962376555267,-0.848044693589282));
#125010=DIRECTION('ref_axis',(-0.736687329167645,-0.420092076143344,-0.529919264233163));
#125011=DIRECTION('center_axis',(0.458928288799633,0.264962371077255,-0.848044673146739));
#125012=DIRECTION('ref_axis',(-0.879478325588519,2.1428654450467E-15,-0.475938940222393));
#125013=DIRECTION('center_axis',(-0.458927817275468,-0.264962073797545,
-0.848045021198568));
#125014=DIRECTION('ref_axis',(0.732266960582963,0.427750712253125,-0.529919264233274));
#125015=DIRECTION('center_axis',(0.458927830768628,0.264962106632877,0.848045003637584));
#125016=DIRECTION('ref_axis',(0.879478602053331,-3.90796687788124E-15,-0.475938429348081));
#125017=DIRECTION('center_axis',(0.499776392786184,-0.866154464985103,-2.36620233737299E-14));
#125018=DIRECTION('ref_axis',(0.866154464985103,0.499776392786184,2.85780049921816E-28));
#125019=DIRECTION('center_axis',(0.86602540378444,0.499999999999998,0.));
#125020=DIRECTION('ref_axis',(-0.499999999999998,0.86602540378444,0.));
#125021=DIRECTION('center_axis',(-1.88658882408992E-17,7.04084534449537E-17,
-1.));
#125022=DIRECTION('ref_axis',(0.,1.,1.20114286872534E-16));
#125023=DIRECTION('center_axis',(0.500223573885301,-0.865896284857152,0.));
#125024=DIRECTION('ref_axis',(0.865896284857152,0.500223573885301,0.));
#125025=DIRECTION('center_axis',(0.866025403784445,0.499999999999989,-1.21951018649011E-16));
#125026=DIRECTION('ref_axis',(-0.499999999999989,0.866025403784445,-1.28346985693928E-30));
#125027=DIRECTION('center_axis',(0.75000880237976,0.432983094186958,-0.500012436346502));
#125028=DIRECTION('ref_axis',(0.432528431881907,0.250863215138471,0.866017784404089));
#125029=DIRECTION('center_axis',(-0.458928288799653,-0.26496237107725,0.84804467314673));
#125030=DIRECTION('ref_axis',(0.879478325588507,4.12607120826034E-15,0.475938940222415));
#125031=DIRECTION('center_axis',(-0.43301703527827,-0.250002513554088,0.866022511471529));
#125032=DIRECTION('ref_axis',(-0.747751775424576,-0.436883602747219,-0.500000000000005));
#125033=DIRECTION('center_axis',(0.433017051950193,0.250002511507141,-0.866022503726367));
#125034=DIRECTION('ref_axis',(-0.894424794863831,4.51772688567625E-15,-0.447218387740032));
#125035=DIRECTION('center_axis',(-0.458928247653241,-0.264962376527612,
0.848044693710636));
#125036=DIRECTION('ref_axis',(-0.732154074453982,-0.427943903631124,-0.529919264233136));
#125037=DIRECTION('center_axis',(-0.458928232223214,-0.264962338412753,
0.848044713969329));
#125038=DIRECTION('ref_axis',(0.879478359737742,3.73673734303752E-16,0.475938877118702));
#125039=DIRECTION('center_axis',(0.86602540378444,0.499999999999998,3.36577552674943E-14));
#125040=DIRECTION('ref_axis',(-0.499999999999998,0.86602540378444,4.57373621403242E-28));
#125041=DIRECTION('center_axis',(-0.866025403784433,-0.50000000000001,0.));
#125042=DIRECTION('ref_axis',(0.50000000000001,-0.866025403784433,0.));
#125043=DIRECTION('center_axis',(0.866025403784445,0.499999999999989,-1.21951018649011E-16));
#125044=DIRECTION('ref_axis',(-0.499999999999989,0.866025403784445,-1.28346985693928E-30));
#125045=DIRECTION('center_axis',(0.86602540378444,0.499999999999998,-2.73184799366421E-14));
#125046=DIRECTION('ref_axis',(-0.499999999999998,0.86602540378444,-3.72554280132519E-28));
#125047=DIRECTION('center_axis',(0.866025403784445,0.499999999999989,-1.21951018649011E-16));
#125048=DIRECTION('ref_axis',(-0.499999999999989,0.866025403784445,-1.28346985693928E-30));
#125049=DIRECTION('center_axis',(-0.750027562856474,-0.432988827019046,
-0.499979330205008));
#125050=DIRECTION('ref_axis',(0.433476564273207,0.249154705651457,-0.866036951219538));
#125051=DIRECTION('center_axis',(0.433017169313169,0.250002579266687,0.866022425483321));
#125052=DIRECTION('ref_axis',(0.894424730216444,-7.57227756159649E-15,-0.447218517033052));
#125053=DIRECTION('center_axis',(0.433017177087304,0.250002583755051,0.866022420300503));
#125054=DIRECTION('ref_axis',(0.499999999999399,-0.866025403784786,3.84644196595208E-13));
#125055=DIRECTION('center_axis',(-0.456777309670065,-0.203370361063163,
0.866022508721116));
#125056=DIRECTION('ref_axis',(-0.406736643075047,0.913545457642936,4.54579507195795E-13));
#125057=DIRECTION('center_axis',(-0.791134794601669,-0.352268789800729,
0.500012436348242));
#125058=DIRECTION('ref_axis',(0.457186437801428,0.202469153670706,0.866017784403016));
#125059=DIRECTION('center_axis',(0.456777317573273,0.203370364581918,-0.866022503726308));
#125060=DIRECTION('ref_axis',(-0.884507036382097,-5.7553372295389E-15,-0.466526850878445));
#125061=DIRECTION('center_axis',(0.913545457642598,0.406736643075807,0.));
#125062=DIRECTION('ref_axis',(-0.406736643075807,0.913545457642598,0.));
#125063=DIRECTION('center_axis',(-0.913545457642606,-0.406736643075789,
1.2864264564856E-16));
#125064=DIRECTION('ref_axis',(0.406736643075789,-0.913545457642606,1.48709352463992E-32));
#125065=DIRECTION('center_axis',(-0.913545457642598,-0.406736643075807,
-1.11114268233636E-14));
#125066=DIRECTION('ref_axis',(0.406736643075807,-0.913545457642598,1.92826049468501E-31));
#125067=DIRECTION('center_axis',(-0.913545457642606,-0.406736643075789,
1.2864264564856E-16));
#125068=DIRECTION('ref_axis',(0.406736643075789,-0.913545457642606,1.48709352463992E-32));
#125069=DIRECTION('center_axis',(0.913545457642598,0.406736643075807,0.));
#125070=DIRECTION('ref_axis',(-0.406736643075807,0.913545457642598,0.));
#125071=DIRECTION('center_axis',(-0.484109857923765,-0.215539595588304,
-0.84804500363758));
#125072=DIRECTION('ref_axis',(-0.868458021515998,-1.76836178502353E-15,
0.495762710240009));
#125073=DIRECTION('center_axis',(0.456777441376074,0.20337041970247,0.866022425483295));
#125074=DIRECTION('ref_axis',(0.884506966812058,2.53897267290044E-15,-0.466526982779059));
#125075=DIRECTION('center_axis',(0.484109840901723,0.215539564337118,0.848045021297498));
#125076=DIRECTION('ref_axis',(0.776473315749238,0.340990855191042,-0.52991926423321));
#125077=DIRECTION('center_axis',(-0.484109806651279,-0.215539572760323,
-0.848045038708652));
#125078=DIRECTION('ref_axis',(-0.868458052949962,-1.14722910183595E-15,
0.495762655175196));
#125079=DIRECTION('center_axis',(0.456777458308629,0.203370415727499,0.866022417485791));
#125080=DIRECTION('ref_axis',(0.792992726927746,0.348084091908492,-0.499999999999938));
#125081=DIRECTION('center_axis',(0.791150459692712,0.352280597671149,0.499979330205228));
#125082=DIRECTION('ref_axis',(0.456361522792999,0.204240445643489,-0.866036951219406));
#125083=DIRECTION('center_axis',(0.406515100163541,-0.913644062717548,0.));
#125084=DIRECTION('ref_axis',(0.913644062717548,0.406515100163541,0.));
#125085=DIRECTION('center_axis',(-0.913545457642606,-0.406736643075789,
1.2864264564856E-16));
#125086=DIRECTION('ref_axis',(0.406736643075789,-0.913545457642606,1.48709352463992E-32));
#125087=DIRECTION('center_axis',(0.913545457642618,0.406736643075761,0.));
#125088=DIRECTION('ref_axis',(-0.406736643075761,0.913545457642618,0.));
#125089=DIRECTION('center_axis',(-1.2174261241351E-17,5.72753959967181E-17,
-1.));
#125090=DIRECTION('ref_axis',(0.,1.,1.12832121675104E-16));
#125091=DIRECTION('center_axis',(0.406958162070199,-0.913446798847336,0.));
#125092=DIRECTION('ref_axis',(0.913446798847336,0.406958162070199,0.));
#125093=DIRECTION('center_axis',(0.484110281406754,0.215539784135092,-0.8480447139693));
#125094=DIRECTION('ref_axis',(-0.868457761888264,-2.53993026454612E-15,
-0.495763165045596));
#125095=DIRECTION('center_axis',(0.484109806651376,0.215539572760315,0.848045038708598));
#125096=DIRECTION('ref_axis',(0.868458052949906,2.93749497420107E-15,-0.495762655175295));
#125097=DIRECTION('center_axis',(0.484110300945566,0.215539820435717,-0.848044693589278));
#125098=DIRECTION('ref_axis',(-0.776563258037241,-0.340785973392545,-0.529919264233223));
#125099=DIRECTION('center_axis',(0.484110341087594,0.215539810706745,-0.848044673146736));
#125100=DIRECTION('ref_axis',(-0.868457725299277,3.13556863905275E-15,-0.495763229140692));
#125101=DIRECTION('center_axis',(-0.484109841074426,-0.215539564338561,
-0.848045021198543));
#125102=DIRECTION('ref_axis',(0.772967650152,0.348864709039245,-0.529919264233202));
#125103=DIRECTION('center_axis',(0.484109857923745,0.215539595588295,0.848045003637594));
#125104=DIRECTION('ref_axis',(0.868458021516011,-2.89436985092629E-15,-0.495762710239986));
#125105=DIRECTION('center_axis',(0.406500770236715,-0.913650438514073,-2.74957490176846E-15));
#125106=DIRECTION('ref_axis',(0.913650438514073,0.406500770236715,5.03959061829502E-30));
#125107=DIRECTION('center_axis',(0.913545457642598,0.406736643075807,4.99133465116398E-14));
#125108=DIRECTION('ref_axis',(-0.406736643075807,0.913545457642598,-2.82923979546378E-31));
#125109=DIRECTION('center_axis',(-1.2174261241351E-17,5.72753959967181E-17,
-1.));
#125110=DIRECTION('ref_axis',(0.,1.,0.));
#125111=DIRECTION('center_axis',(0.406972488803016,-0.913440415876963,-2.71806413419201E-15));
#125112=DIRECTION('ref_axis',(0.913440415876963,0.406972488803016,-2.33723455769851E-29));
#125113=DIRECTION('center_axis',(0.913545457642606,0.406736643075789,-1.2864264564856E-16));
#125114=DIRECTION('ref_axis',(-0.406736643075789,0.913545457642606,-2.52138284268272E-30));
#125115=DIRECTION('center_axis',(0.791159233140775,0.352213899940326,-0.500012436350263));
#125116=DIRECTION('ref_axis',(0.456381342221735,0.204277427954193,0.86601778440186));
#125117=DIRECTION('center_axis',(-0.484110341087625,-0.215539810706664,
0.848044673146739));
#125118=DIRECTION('ref_axis',(0.868457725299263,1.28125800661297E-15,0.495763229140715));
#125119=DIRECTION('center_axis',(-0.456777301206709,-0.203370368359864,
0.866022511471549));
#125120=DIRECTION('ref_axis',(-0.789322284582009,-0.356328964669238,-0.499999999999987));
#125121=DIRECTION('center_axis',(0.456777317573189,0.203370364581875,-0.866022503726362));
#125122=DIRECTION('ref_axis',(-0.884507036382145,-1.64379723448746E-15,
-0.466526850878354));
#125123=DIRECTION('center_axis',(-0.484110300736294,-0.215539820428334,
0.848044693710618));
#125124=DIRECTION('ref_axis',(-0.772875576443094,-0.349068641863358,-0.529919264233171));
#125125=DIRECTION('center_axis',(-0.484110281406742,-0.215539784135016,
0.848044713969326));
#125126=DIRECTION('ref_axis',(0.868457761888277,-2.39045094596213E-15,0.495763165045575));
#125127=DIRECTION('center_axis',(0.913545457642598,0.406736643075807,1.11114268233636E-14));
#125128=DIRECTION('ref_axis',(-0.406736643075807,0.913545457642598,-1.92826049468501E-31));
#125129=DIRECTION('center_axis',(-0.913545457642594,-0.406736643075817,
0.));
#125130=DIRECTION('ref_axis',(0.406736643075817,-0.913545457642593,0.));
#125131=DIRECTION('center_axis',(0.913545457642606,0.406736643075789,-1.2864264564856E-16));
#125132=DIRECTION('ref_axis',(-0.406736643075789,0.913545457642606,-2.52138284268272E-30));
#125133=DIRECTION('center_axis',(0.913545457642598,0.406736643075807,-6.10247733350034E-14));
#125134=DIRECTION('ref_axis',(-0.406736643075807,0.913545457642598,1.41175456657023E-30));
#125135=DIRECTION('center_axis',(0.913545457642606,0.406736643075789,-1.2864264564856E-16));
#125136=DIRECTION('ref_axis',(-0.406736643075789,0.913545457642606,-2.52138284268272E-30));
#125137=DIRECTION('center_axis',(-0.791178490090679,-0.352217640366629,
-0.499979330205157));
#125138=DIRECTION('ref_axis',(0.457145692795638,0.202479170980401,-0.866036951219453));
#125139=DIRECTION('center_axis',(0.45677744137607,0.203370419702469,0.866022425483297));
#125140=DIRECTION('ref_axis',(0.884506966812061,-6.18778487782607E-15,-0.466526982779054));
#125141=DIRECTION('center_axis',(0.456777449578343,0.203370423354363,0.866022420299481));
#125142=DIRECTION('ref_axis',(0.406736643083121,-0.913545457639341,-4.61573035911191E-12));
#125143=DIRECTION('center_axis',(-0.475533027090268,-0.154510046710891,
0.866022508721202));
#125144=DIRECTION('ref_axis',(-0.30901699437301,0.951056516295783,1.18890024959428E-12));
#125145=DIRECTION('center_axis',(-0.823622990673951,-0.267642920194547,
0.50001243634837));
#125146=DIRECTION('ref_axis',(0.475845712142861,0.153571010718269,0.866017784402967));
#125147=DIRECTION('center_axis',(0.475533035318122,0.154510049384294,-0.866022503726316));
#125148=DIRECTION('ref_axis',(-0.876548788012445,9.99951496082734E-16,-0.48131301897405));
#125149=DIRECTION('center_axis',(0.951056516295165,0.309016994374914,-6.04047112789571E-14));
#125150=DIRECTION('ref_axis',(-0.309016994374914,0.951056516295164,-2.46817372928747E-30));
#125151=DIRECTION('center_axis',(-0.951056516295158,-0.309016994374935,
1.33924836902178E-16));
#125152=DIRECTION('ref_axis',(0.309016994374935,-0.951056516295158,-9.27809067577952E-33));
#125153=DIRECTION('center_axis',(-0.951056516295165,-0.309016994374914,
-5.19628367180445E-14));
#125154=DIRECTION('ref_axis',(0.309016994374914,-0.951056516295164,-1.42492764277297E-30));
#125155=DIRECTION('center_axis',(-0.951056516295158,-0.309016994374935,
1.33924836902178E-16));
#125156=DIRECTION('ref_axis',(0.309016994374935,-0.951056516295158,3.04786096829879E-33));
#125157=DIRECTION('center_axis',(0.951056516295165,0.309016994374914,0.));
#125158=DIRECTION('ref_axis',(-0.309016994374914,0.951056516295164,0.));
#125159=DIRECTION('center_axis',(-0.503987876168997,-0.163755587629879,
-0.848045003637577));
#125160=DIRECTION('ref_axis',(-0.859649462041482,-2.31443907975747E-15,
0.510884333691875));
#125161=DIRECTION('center_axis',(0.475533164204451,0.15451009126196,0.866022425483269));
#125162=DIRECTION('ref_axis',(0.876548714628815,1.61550628132638E-15,-0.481313152617475));
#125163=DIRECTION('center_axis',(0.503987855974665,0.163755558325779,0.848045021297497));
#125164=DIRECTION('ref_axis',(0.807862963764707,0.257959309139721,-0.529919264233205));
#125165=DIRECTION('center_axis',(-0.503987822791223,-0.163755570286389,
-0.848045038708642));
#125166=DIRECTION('ref_axis',(-0.859649495083692,-4.55730791939964E-15,
0.510884278092753));
#125167=DIRECTION('center_axis',(0.475533180627103,0.154510085543892,0.866022417485766));
#125168=DIRECTION('ref_axis',(0.825033325009168,0.263286939714686,-0.499999999999991));
#125169=DIRECTION('center_axis',(0.82363980420873,0.267653025932129,0.499979330205139));
#125170=DIRECTION('ref_axis',(0.475210466543398,0.155418826433942,-0.866036951219463));
#125171=DIRECTION('center_axis',(0.308786358060973,-0.951131423661021,2.59834647143935E-14));
#125172=DIRECTION('ref_axis',(0.951131423661021,0.308786358060973,1.96167695623581E-28));
#125173=DIRECTION('center_axis',(-0.951056516295158,-0.309016994374935,
1.33924836902178E-16));
#125174=DIRECTION('ref_axis',(0.309016994374935,-0.951056516295158,-9.27809067577952E-33));
#125175=DIRECTION('center_axis',(0.951056516295165,0.309016994374914,0.));
#125176=DIRECTION('ref_axis',(-0.309016994374914,0.951056516295164,0.));
#125177=DIRECTION('center_axis',(-6.89206998773264E-18,4.35148173242952E-17,
-1.));
#125178=DIRECTION('ref_axis',(0.,1.,0.));
#125179=DIRECTION('center_axis',(0.309247612517378,-0.95098155300316,0.));
#125180=DIRECTION('ref_axis',(0.95098155300316,0.309247612517378,0.));
#125181=DIRECTION('center_axis',(0.503988317040571,0.163755730877732,-0.848044713969324));
#125182=DIRECTION('ref_axis',(-0.859649189130473,-1.51298268767331E-15,
-0.510884792910614));
#125183=DIRECTION('center_axis',(0.503987822791218,0.163755570286387,0.848045038708645));
#125184=DIRECTION('ref_axis',(0.859649495083696,-2.0335524798323E-15,-0.510884278092747));
#125185=DIRECTION('center_axis',(0.503988340265571,0.163755764941051,-0.848044693589274));
#125186=DIRECTION('ref_axis',(-0.807930997363437,-0.257746148165048,-0.52991926423315));
#125187=DIRECTION('center_axis',(0.503988379172015,0.163755751065486,-0.84804467314673));
#125188=DIRECTION('ref_axis',(-0.859649150669458,-3.94104971099401E-15,
-0.510884857627704));
#125189=DIRECTION('center_axis',(-0.503987856144593,-0.163755558315073,
-0.848045021198578));
#125190=DIRECTION('ref_axis',(0.805199544413242,0.266156471030219,-0.529919264233193));
#125191=DIRECTION('center_axis',(0.503987876168979,0.163755587629873,0.848045003637589));
#125192=DIRECTION('ref_axis',(0.859649462041493,-1.78492124839558E-15,-0.510884333691856));
#125193=DIRECTION('center_axis',(0.308771440182783,-0.951136266645033,-9.11326423007215E-15));
#125194=DIRECTION('ref_axis',(0.951136266645033,0.308771440182783,2.771149958367E-29));
#125195=DIRECTION('center_axis',(0.951056516295165,0.309016994374914,8.44187456091256E-15));
#125196=DIRECTION('ref_axis',(-0.309016994374914,0.951056516295164,1.39291926319097E-31));
#125197=DIRECTION('center_axis',(-6.89206998773264E-18,4.35148173242952E-17,
-1.));
#125198=DIRECTION('ref_axis',(0.,1.,0.));
#125199=DIRECTION('center_axis',(0.309262527968943,-0.95097670255073,0.));
#125200=DIRECTION('ref_axis',(0.950976702550729,0.309262527968943,0.));
#125201=DIRECTION('center_axis',(0.951056516295158,0.309016994374935,-1.33924836902178E-16));
#125202=DIRECTION('ref_axis',(-0.309016994374935,0.951056516295158,2.92272947789642E-30));
#125203=DIRECTION('center_axis',(0.823641557784016,0.267585776504269,-0.500012436349064));
#125204=DIRECTION('ref_axis',(0.475234043092174,0.155453534487958,0.86601778440253));
#125205=DIRECTION('center_axis',(-0.503988379172015,-0.163755751065433,
0.84804467314674));
#125206=DIRECTION('ref_axis',(0.859649150669461,4.80415871610856E-15,0.510884857627699));
#125207=DIRECTION('center_axis',(-0.475533019436127,-0.154510054852395,
0.866022511471538));
#125208=DIRECTION('ref_axis',(-0.822244813612915,-0.271870311889065,-0.500000000000005));
#125209=DIRECTION('center_axis',(0.475533035318005,0.15451004938422,-0.866022503726394));
#125210=DIRECTION('ref_axis',(-0.876548788012513,-2.02407478928591E-15,
-0.481313018973926));
#125211=DIRECTION('center_axis',(-0.503988340058875,-0.163755764948789,
0.848044693710618));
#125212=DIRECTION('ref_axis',(-0.805129291879029,-0.266368911010517,-0.529919264233189));
#125213=DIRECTION('center_axis',(-0.503988317040557,-0.163755730877752,
0.848044713969329));
#125214=DIRECTION('ref_axis',(0.85964918913048,3.98009309471949E-15,0.510884792910601));
#125215=DIRECTION('center_axis',(0.951056516295165,0.309016994374914,-6.04047112789571E-14));
#125216=DIRECTION('ref_axis',(-0.309016994374914,0.951056516295164,-2.46817372928747E-30));
#125217=DIRECTION('center_axis',(-0.951056516295165,-0.309016994374914,
0.));
#125218=DIRECTION('ref_axis',(0.309016994374914,-0.951056516295164,0.));
#125219=DIRECTION('center_axis',(0.951056516295158,0.309016994374935,-1.33924836902178E-16));
#125220=DIRECTION('ref_axis',(-0.309016994374935,0.951056516295158,2.92272947789642E-30));
#125221=DIRECTION('center_axis',(0.951056516295165,0.309016994374914,-4.3520962157132E-14));
#125222=DIRECTION('ref_axis',(-0.309016994374914,0.951056516295164,-1.2145041730042E-30));
#125223=DIRECTION('center_axis',(0.951056516295158,0.309016994374935,-1.33924836902178E-16));
#125224=DIRECTION('ref_axis',(-0.309016994374935,0.951056516295158,2.92272947789642E-30));
#125225=DIRECTION('center_axis',(-0.823661100222713,-0.267587483540128,
-0.499979330205332));
#125226=DIRECTION('ref_axis',(0.47580623744722,0.153585232131932,-0.866036951219346));
#125227=DIRECTION('center_axis',(0.475533164204429,0.154510091261957,0.866022425483281));
#125228=DIRECTION('ref_axis',(0.876548714628827,1.44586213632941E-15,-0.481313152617453));
#125229=DIRECTION('center_axis',(0.475533172742431,0.154510094036134,0.866022420300111));
#125230=DIRECTION('ref_axis',(0.309016994376992,-0.951056516294489,-1.25883555248922E-12));
#125231=DIRECTION('center_axis',(-0.48907870515122,-0.103956887952953,0.866022508722922));
#125232=DIRECTION('ref_axis',(-0.207911690817661,0.978147600733827,6.99353087993298E-14));
#125233=DIRECTION('center_axis',(-0.847087400905761,-0.180084698747582,
0.500012436349052));
#125234=DIRECTION('ref_axis',(0.489291521290444,0.102990311639969,0.866017784402598));
#125235=DIRECTION('center_axis',(0.489078713616366,0.103956889752291,-0.866022503726313));
#125236=DIRECTION('ref_axis',(-0.870740345484705,-2.30898284559697E-15,
-0.491743073916834));
#125237=DIRECTION('center_axis',(0.978147600733806,0.207911690817757,0.));
#125238=DIRECTION('ref_axis',(-0.207911690817757,0.978147600733806,0.));
#125239=DIRECTION('center_axis',(-0.978147600733808,-0.207911690817747,
1.37739719617122E-16));
#125240=DIRECTION('ref_axis',(0.207911690817747,-0.978147600733808,-5.77321332412281E-33));
#125241=DIRECTION('center_axis',(-0.978147600733807,-0.207911690817754,
-2.83991567709909E-15));
#125242=DIRECTION('ref_axis',(0.207911690817754,-0.978147600733807,-8.10663864458446E-30));
#125243=DIRECTION('center_axis',(-0.978147600733808,-0.207911690817747,
1.37739719617122E-16));
#125244=DIRECTION('ref_axis',(0.207911690817747,-0.978147600733808,1.27157141419947E-32));
#125245=DIRECTION('center_axis',(0.978147600733806,0.207911690817757,0.));
#125246=DIRECTION('ref_axis',(-0.207911690817757,0.978147600733806,0.));
#125247=DIRECTION('center_axis',(-0.518344097776651,-0.110177439185352,
-0.848045003637583));
#125248=DIRECTION('ref_axis',(-0.85323958281187,2.74380692439891E-15,0.521519140898036));
#125249=DIRECTION('center_axis',(0.489078846174035,0.103956917928313,0.866022425483267));
#125250=DIRECTION('ref_axis',(0.870740269393757,1.63311310360591E-16,-0.491743208652736));
#125251=DIRECTION('center_axis',(0.518344074628942,0.110177412156896,0.848045021297499));
#125252=DIRECTION('ref_axis',(0.830401496088695,0.172101506931704,-0.529919264233235));
#125253=DIRECTION('center_axis',(-0.518344042878405,-0.11017742751637,-0.848045038708644));
#125254=DIRECTION('ref_axis',(-0.853239616987299,-4.34819448574131E-16,
0.521519084984785));
#125255=DIRECTION('center_axis',(0.489078861909502,0.103956910522811,0.866022417485748));
#125256=DIRECTION('ref_axis',(0.84803468533791,0.1756051606982,-0.499999999999992));
#125257=DIRECTION('center_axis',(0.847105178672016,0.180092991630677,0.499979330205324));
#125258=DIRECTION('ref_axis',(0.488852904975635,0.104894406045156,-0.866036951219356));
#125259=DIRECTION('center_axis',(0.207674488001815,-0.978197989689809,0.));
#125260=DIRECTION('ref_axis',(0.978197989689809,0.207674488001815,0.));
#125261=DIRECTION('center_axis',(-0.978147600733808,-0.207911690817747,
1.37739719617122E-16));
#125262=DIRECTION('ref_axis',(0.207911690817747,-0.978147600733808,-5.77321332412281E-33));
#125263=DIRECTION('center_axis',(0.978147600733806,0.207911690817757,0.));
#125264=DIRECTION('ref_axis',(-0.207911690817757,0.978147600733806,0.));
#125265=DIRECTION('center_axis',(-3.07718727278846E-18,2.92774812072065E-17,
-1.));
#125266=DIRECTION('ref_axis',(0.,1.,0.));
#125267=DIRECTION('center_axis',(0.208148881407602,-0.978097154258596,0.));
#125268=DIRECTION('ref_axis',(0.978097154258596,0.208148881407602,0.));
#125269=DIRECTION('center_axis',(0.518344551206563,0.110177535564868,-0.848044713969328));
#125270=DIRECTION('ref_axis',(-0.853239300541053,2.15107083335551E-15,-0.52151960271136));
#125271=DIRECTION('center_axis',(0.51834404287839,0.110177427516366,0.848045038708654));
#125272=DIRECTION('ref_axis',(0.853239616987309,-2.70652115665923E-15,-0.521519084984769));
#125273=DIRECTION('center_axis',(0.518344577867921,0.110177566999581,-0.848044693589306));
#125274=DIRECTION('ref_axis',(-0.830446875599428,-0.171882402245342,-0.529919264233259));
#125275=DIRECTION('center_axis',(0.518344615107839,0.110177549147491,-0.848044673146738));
#125276=DIRECTION('ref_axis',(-0.853239260760973,3.52957760131147E-15,-0.5215196677941));
#125277=DIRECTION('center_axis',(-0.51834407479893,-0.110177412118683,-0.848045021198563));
#125278=DIRECTION('ref_axis',(0.828609503964271,0.180532167035843,-0.529919264233173));
#125279=DIRECTION('center_axis',(0.518344097776644,0.11017743918535,0.848045003637587));
#125280=DIRECTION('ref_axis',(0.853239582811874,-1.85602097405422E-15,-0.52151914089803));
#125281=DIRECTION('center_axis',(0.207659145615641,-0.978201246800566,0.));
#125282=DIRECTION('ref_axis',(0.978201246800566,0.207659145615641,0.));
#125283=DIRECTION('center_axis',(0.978147600733807,0.207911690817754,0.));
#125284=DIRECTION('ref_axis',(-0.207911690817754,0.978147600733807,0.));
#125285=DIRECTION('center_axis',(-3.07718727278846E-18,2.92774812072065E-17,
-1.));
#125286=DIRECTION('ref_axis',(0.,1.,0.));
#125287=DIRECTION('center_axis',(0.208164222161082,-0.978093889466687,1.13734602532685E-14));
#125288=DIRECTION('ref_axis',(0.978093889466687,0.208164222161082,4.2991390833162E-29));
#125289=DIRECTION('center_axis',(0.978147600733808,0.207911690817747,-1.37739719617122E-16));
#125290=DIRECTION('ref_axis',(-0.207911690817747,0.978147600733808,-1.05212114846847E-30));
#125291=DIRECTION('center_axis',(0.847099893161591,0.180025927304202,-0.500012436349221));
#125292=DIRECTION('ref_axis',(0.488879980351705,0.104926459532324,0.86601778440245));
#125293=DIRECTION('center_axis',(-0.518344615107841,-0.110177549147463,
0.848044673146741));
#125294=DIRECTION('ref_axis',(0.853239260760973,-3.53605500348288E-15,0.5215196677941));
#125295=DIRECTION('center_axis',(-0.489078698392428,-0.103956896852848,
0.866022511471552));
#125296=DIRECTION('ref_axis',(-0.846158656400491,-0.184432991079564,-0.499999999999962));
#125297=DIRECTION('center_axis',(0.489078713616248,0.103956889752265,-0.866022503726382));
#125298=DIRECTION('ref_axis',(-0.870740345484772,1.04734835562025E-15,-0.491743073916714));
#125299=DIRECTION('center_axis',(-0.51834457766095,-0.110177567039741,0.848044693710594));
#125300=DIRECTION('ref_axis',(-0.82856184230912,-0.180750786620166,-0.529919264233249));
#125301=DIRECTION('center_axis',(-0.518344551206586,-0.110177535564814,
0.848044713969321));
#125302=DIRECTION('ref_axis',(0.85323930054104,3.44800433278326E-15,0.521519602711381));
#125303=DIRECTION('center_axis',(0.978147600733807,0.207911690817754,0.));
#125304=DIRECTION('ref_axis',(-0.207911690817754,0.978147600733807,0.));
#125305=DIRECTION('center_axis',(-0.978147600733807,-0.207911690817754,
0.));
#125306=DIRECTION('ref_axis',(0.207911690817754,-0.978147600733807,0.));
#125307=DIRECTION('center_axis',(0.978147600733808,0.207911690817747,-1.37739719617122E-16));
#125308=DIRECTION('ref_axis',(-0.207911690817747,0.978147600733808,-1.05212114846847E-30));
#125309=DIRECTION('center_axis',(0.978147600733807,0.207911690817754,5.34430112114424E-14));
#125310=DIRECTION('ref_axis',(-0.207911690817754,0.978147600733807,1.52655727061559E-28));
#125311=DIRECTION('center_axis',(0.978147600733808,0.207911690817747,-1.37739719617122E-16));
#125312=DIRECTION('ref_axis',(-0.207911690817747,0.978147600733808,-1.05212114846847E-30));
#125313=DIRECTION('center_axis',(-0.847119506978902,-0.180025582247299,
-0.499979330205103));
#125314=DIRECTION('ref_axis',(0.489253749387821,0.103008581353307,-0.866036951219484));
#125315=DIRECTION('center_axis',(0.489078846174003,0.103956917928285,0.866022425483288));
#125316=DIRECTION('ref_axis',(0.870740269393775,-7.78986752012561E-16,-0.491743208652702));
#125317=DIRECTION('center_axis',(0.489078854943167,0.103956919792226,0.86602242030723));
#125318=DIRECTION('ref_axis',(0.207911690809382,-0.978147600735586,4.93043924728801E-12));
#125319=DIRECTION('center_axis',(-0.497265934578102,-0.0522647557774919,
0.866022508721157));
#125320=DIRECTION('ref_axis',(-0.104528463268414,0.994521895368193,-4.54579507199312E-13));
#125321=DIRECTION('center_axis',(-0.861270944309288,-0.0905534316550128,
0.500012436349425));
#125322=DIRECTION('ref_axis',(0.497376550150498,0.0512812291116259,0.86601778440237));
#125323=DIRECTION('center_axis',(0.497265943181925,0.0522647566817413,-0.866022503726311));
#125324=DIRECTION('ref_axis',(-0.867207748104374,-9.26225114799316E-16,
-0.497946504785143));
#125325=DIRECTION('center_axis',(0.994521895368276,0.104528463267629,0.));
#125326=DIRECTION('ref_axis',(-0.104528463267629,0.994521895368276,0.));
#125327=DIRECTION('center_axis',(-0.994521895368275,-0.10452846326764,1.40045497140052E-16));
#125328=DIRECTION('ref_axis',(0.10452846326764,-0.994521895368275,-1.79838028938001E-33));
#125329=DIRECTION('center_axis',(-0.994521895368276,-0.104528463267629,
0.));
#125330=DIRECTION('ref_axis',(0.104528463267629,-0.994521895368276,0.));
#125331=DIRECTION('center_axis',(-0.994521895368275,-0.10452846326764,1.40045497140052E-16));
#125332=DIRECTION('ref_axis',(0.10452846326764,-0.994521895368275,-1.79838028938001E-33));
#125333=DIRECTION('center_axis',(0.994521895368276,0.10452846326763,0.));
#125334=DIRECTION('ref_axis',(-0.10452846326763,0.994521895368276,0.));
#125335=DIRECTION('center_axis',(-0.527021232978627,-0.0553921636609794,
-0.848045003637568));
#125336=DIRECTION('ref_axis',(-0.849349030019368,-1.01561542645059E-15,
0.527831625809934));
#125337=DIRECTION('center_axis',(0.497266077958573,0.0522647708473857,0.866022425483295));
#125338=DIRECTION('ref_axis',(0.867207670398082,3.99694090177787E-16,-0.497946640115919));
#125339=DIRECTION('center_axis',(0.527021207132431,0.0553921392005086,0.848045021297494));
#125340=DIRECTION('ref_axis',(0.843841975852503,0.084358124587104,-0.529919264233232));
#125341=DIRECTION('center_axis',(-0.527021177161347,-0.0553921577943469,
-0.848045038708649));
#125342=DIRECTION('ref_axis',(-0.849349064867519,-4.73002354866103E-16,
0.527831569734769));
#125343=DIRECTION('center_axis',(0.49726609283361,0.0522647618391874,0.866022417485765));
#125344=DIRECTION('ref_axis',(0.861744800189585,0.0859994148015332,-0.500000000000005));
#125345=DIRECTION('center_axis',(0.861289491529721,0.090559820826828,0.499979330205046));
#125346=DIRECTION('ref_axis',(0.497139368682281,0.0532207405865388,-0.866036951219521));
#125347=DIRECTION('center_axis',(0.104287292793425,-0.994547213842469,0.));
#125348=DIRECTION('ref_axis',(0.994547213842469,0.104287292793425,0.));
#125349=DIRECTION('center_axis',(-0.994521895368275,-0.10452846326764,1.40045497140052E-16));
#125350=DIRECTION('ref_axis',(0.10452846326764,-0.994521895368275,-1.79838028938001E-33));
#125351=DIRECTION('center_axis',(0.994521895368276,0.10452846326763,0.));
#125352=DIRECTION('ref_axis',(-0.10452846326763,0.994521895368276,0.));
#125353=DIRECTION('center_axis',(-7.71409749858844E-19,1.47193748793047E-17,
-1.));
#125354=DIRECTION('ref_axis',(0.,1.,0.));
#125355=DIRECTION('center_axis',(0.104769627595152,-0.994496518411992,0.));
#125356=DIRECTION('ref_axis',(0.994496518411992,0.104769627595152,0.));
#125357=DIRECTION('center_axis',(0.527021693999021,0.0553922121161754,-0.848044713969304));
#125358=DIRECTION('ref_axis',(-0.849348742192388,1.01528730975471E-15,-0.527832088960314));
#125359=DIRECTION('center_axis',(0.527021177161445,0.0553921577943106,0.848045038708591));
#125360=DIRECTION('ref_axis',(0.849349064867459,8.87709183645612E-16,-0.527831569734866));
#125361=DIRECTION('center_axis',(0.527021723799587,0.0553922405971153,-0.848044693589284));
#125362=DIRECTION('ref_axis',(-0.843864204095477,-0.0841354767077662,-0.529919264233208));
#125363=DIRECTION('center_axis',(0.527021758969976,0.0553922189448975,-0.848044673146735));
#125364=DIRECTION('ref_axis',(-0.849348701629308,-8.38249277152437E-16,
-0.527832154231445));
#125365=DIRECTION('center_axis',(-0.527021207296642,-0.0553921391525556,
-0.848045021198577));
#125366=DIRECTION('ref_axis',(0.842941044396022,0.092929914812537,-0.529919264233221));
#125367=DIRECTION('center_axis',(0.527021232978636,0.0553921636609804,0.848045003637562));
#125368=DIRECTION('ref_axis',(0.849349030019363,4.17709715649168E-16,-0.527831625809943));
#125369=DIRECTION('center_axis',(0.10427169399366,-0.994548849394384,-1.24894790576994E-14));
#125370=DIRECTION('ref_axis',(0.994548849394384,0.10427169399366,-6.77001402833622E-29));
#125371=DIRECTION('center_axis',(0.994521895368276,0.104528463267629,0.));
#125372=DIRECTION('ref_axis',(-0.104528463267629,0.994521895368276,0.));
#125373=DIRECTION('center_axis',(-7.71409749858844E-19,1.47193748793047E-17,
-1.));
#125374=DIRECTION('ref_axis',(0.,1.,0.));
#125375=DIRECTION('center_axis',(0.104785225574074,-0.99449487505034,0.));
#125376=DIRECTION('ref_axis',(0.994494875050339,0.104785225574074,0.));
#125377=DIRECTION('center_axis',(0.994521895368275,0.10452846326764,-1.40045497140052E-16));
#125378=DIRECTION('ref_axis',(-0.10452846326764,0.994521895368275,1.56623842824886E-30));
#125379=DIRECTION('center_axis',(0.861277224843046,0.0904936763733016,-0.500012436348442));
#125380=DIRECTION('ref_axis',(0.497169646239973,0.0532497883138783,0.866017784402923));
#125381=DIRECTION('center_axis',(-0.527021758969983,-0.0553922189448987,
0.848044673146731));
#125382=DIRECTION('ref_axis',(0.849348701629304,3.53735120591045E-16,0.527832154231453));
#125383=DIRECTION('center_axis',(-0.497265928782812,-0.0522647653419817,
0.866022511471564));
#125384=DIRECTION('ref_axis',(-0.860801807878642,-0.0949749838266845,-0.499999999999982));
#125385=DIRECTION('center_axis',(0.497265943181779,0.0522647566817739,-0.866022503726393));
#125386=DIRECTION('ref_axis',(-0.867207748104458,5.79523975621388E-16,-0.497946504784997));
#125387=DIRECTION('center_axis',(-0.527021723597968,-0.055392240657868,
0.848044693710613));
#125388=DIRECTION('ref_axis',(-0.842916495800633,-0.0931523188209939,-0.529919264233198));
#125389=DIRECTION('center_axis',(-0.527021693999002,-0.0553922121161264,
0.848044713969319));
#125390=DIRECTION('ref_axis',(0.849348742192401,3.31432934842991E-16,0.527832088960293));
#125391=DIRECTION('center_axis',(0.994521895368276,0.104528463267629,1.42777936329238E-15));
#125392=DIRECTION('ref_axis',(-0.104528463267629,0.994521895368276,-1.03141617847887E-30));
#125393=DIRECTION('center_axis',(-0.994521895368276,-0.104528463267628,
0.));
#125394=DIRECTION('ref_axis',(0.104528463267628,-0.994521895368276,0.));
#125395=DIRECTION('center_axis',(0.994521895368275,0.10452846326764,-1.40045497140052E-16));
#125396=DIRECTION('ref_axis',(-0.10452846326764,0.994521895368275,1.56623842824886E-30));
#125397=DIRECTION('center_axis',(0.994521895368276,0.104528463267629,-7.13889681646191E-16));
#125398=DIRECTION('ref_axis',(-0.104528463267629,0.994521895368276,5.15708089239434E-31));
#125399=DIRECTION('center_axis',(0.994521895368275,0.10452846326764,-1.40045497140052E-16));
#125400=DIRECTION('ref_axis',(-0.10452846326764,0.994521895368275,1.56623842824886E-30));
#125401=DIRECTION('center_axis',(-0.861296695145335,-0.0904912830026736,
-0.499979330205014));
#125402=DIRECTION('ref_axis',(0.497340894868559,0.0513033470029239,-0.866036951219542));
#125403=DIRECTION('center_axis',(0.497266077958562,0.0522647708473845,0.866022425483301));
#125404=DIRECTION('ref_axis',(0.867207670398088,1.09710147407178E-15,-0.497946640115907));
#125405=DIRECTION('center_axis',(0.497266086887884,0.052264771785901,0.866022420299486));
#125406=DIRECTION('ref_axis',(0.104528463274216,-0.994521895367584,-3.84644196591536E-12));
#125407=DIRECTION('center_axis',(-1.40816906889909E-16,-7.12377958457618E-15,
1.));
#125408=DIRECTION('ref_axis',(0.,-1.,-7.12427864012715E-15));
#125409=DIRECTION('center_axis',(-1.40816906889909E-16,-7.12377958457618E-15,
1.));
#125410=DIRECTION('ref_axis',(-3.91292818132308E-34,-1.,-7.12377958457618E-15));
#125411=DIRECTION('center_axis',(0.99999996667151,-0.00025818012795372,
1.58266350846276E-16));
#125412=DIRECTION('ref_axis',(-0.00025818012795372,-0.99999996667151,-6.82961998416055E-15));
#125413=DIRECTION('center_axis',(1.4081690688991E-16,6.98296267768627E-15,
-1.));
#125414=DIRECTION('ref_axis',(-1.,4.05186995067197E-12,-1.40816906861616E-16));
#125415=DIRECTION('center_axis',(0.99999996667151,0.000258180127974661,
1.35193873067682E-16));
#125416=DIRECTION('ref_axis',(0.000258180127974661,-0.99999996667151,-6.82961998416055E-15));
#125417=DIRECTION('center_axis',(-1.40816906889909E-16,-7.12377958457618E-15,
1.));
#125418=DIRECTION('ref_axis',(0.,-1.,-7.12252768074091E-15));
#125419=DIRECTION('center_axis',(-1.4081690688991E-16,-6.98296267768627E-15,
1.));
#125420=DIRECTION('ref_axis',(1.,-4.31477076290321E-12,1.40816906859781E-16));
#125421=DIRECTION('center_axis',(0.999999970597889,-0.000242495818320685,
1.45036773284196E-16));
#125422=DIRECTION('ref_axis',(-0.000242495818320685,-0.999999970597889,
-6.82961998416057E-15));
#125423=DIRECTION('center_axis',(1.40816906889909E-16,7.12377958457618E-15,
-1.));
#125424=DIRECTION('ref_axis',(9.00435281891987E-12,-1.,-7.12377958457491E-15));
#125425=DIRECTION('center_axis',(0.999999970597889,0.000242495818341616,
1.7510165406073E-16));
#125426=DIRECTION('ref_axis',(0.000242495818341616,-0.999999970597889,-6.82961998416057E-15));
#125427=DIRECTION('center_axis',(-2.81633813779821E-16,-6.98296267768627E-15,
1.));
#125428=DIRECTION('ref_axis',(-1.,2.13365834995709E-30,-2.77764288392734E-16));
#125429=DIRECTION('center_axis',(-2.81633813779821E-16,-6.98296267768627E-15,
1.));
#125430=DIRECTION('ref_axis',(-1.,2.10523536799201E-30,-2.81633813779821E-16));
#125431=DIRECTION('center_axis',(-0.00025818012796419,-0.99999996667151,
-6.98372952115933E-15));
#125432=DIRECTION('ref_axis',(-0.99999996667151,0.00025818012796419,4.97610099109124E-32));
#125433=DIRECTION('center_axis',(1.4081690688991E-16,6.98296267768627E-15,
-1.));
#125434=DIRECTION('ref_axis',(-1.,3.98880928287326E-12,-1.40816906862057E-16));
#125435=DIRECTION('center_axis',(0.00025818012796419,-0.99999996667151,
-6.98219536875E-15));
#125436=DIRECTION('ref_axis',(-0.99999996667151,-0.00025818012796419,-4.98515713638296E-32));
#125437=DIRECTION('center_axis',(-2.81633813779821E-16,-6.98296267768627E-15,
1.));
#125438=DIRECTION('ref_axis',(-1.,2.00430111041611E-30,-2.82080304187759E-16));
#125439=DIRECTION('center_axis',(-1.4081690688991E-16,-6.98296267768627E-15,
1.));
#125440=DIRECTION('ref_axis',(1.,-1.19598452005484E-30,1.4081690688991E-16));
#125441=DIRECTION('center_axis',(-0.000242495818331158,-0.999999970597889,
-6.98296247237242E-15));
#125442=DIRECTION('ref_axis',(-0.999999970597889,0.000242495818331158,5.20911529687998E-32));
#125443=DIRECTION('center_axis',(2.81633813779821E-16,6.98296267768627E-15,
-1.));
#125444=DIRECTION('ref_axis',(-1.,9.2414964569798E-12,-2.81633813715288E-16));
#125445=DIRECTION('center_axis',(0.00024249581833115,-0.999999970597889,
-6.96962337123306E-15));
#125446=DIRECTION('ref_axis',(-0.999999970597889,-0.00024249581833115,-9.17267951536334E-32));
#125447=DIRECTION('center_axis',(-1.4081690688991E-16,-6.98296267768627E-15,
1.));
#125448=DIRECTION('ref_axis',(1.,-1.19598452005484E-30,1.4081690688991E-16));
#125449=DIRECTION('center_axis',(-1.4081690688991E-16,-6.98296267768627E-15,
1.));
#125450=DIRECTION('ref_axis',(-1.,8.57836796235549E-31,-1.35821020636094E-16));
#125451=DIRECTION('center_axis',(-1.4081690688991E-16,-6.98296267768627E-15,
1.));
#125452=DIRECTION('ref_axis',(-1.,8.41864228189078E-31,-1.4081690688991E-16));
#125453=DIRECTION('center_axis',(-1.22464679914736E-16,1.,6.98296267768627E-15));
#125454=DIRECTION('ref_axis',(1.,1.22464679914735E-16,1.41480229829265E-16));
#125455=DIRECTION('center_axis',(1.4081690688991E-16,6.98296267768627E-15,
-1.));
#125456=DIRECTION('ref_axis',(-1.,8.40543590285906E-31,-1.4081690688991E-16));
#125457=DIRECTION('center_axis',(1.4081690688991E-16,6.98296267768627E-15,
-1.));
#125458=DIRECTION('ref_axis',(-1.,8.40543590285906E-31,-1.4081690688991E-16));
#125459=DIRECTION('center_axis',(-1.4081690688991E-16,-6.98296267768627E-15,
1.));
#125460=DIRECTION('ref_axis',(-1.,8.5653263190156E-31,-1.3561453272173E-16));
#125461=DIRECTION('center_axis',(-1.4081690688991E-16,-6.98296267768627E-15,
1.));
#125462=DIRECTION('ref_axis',(1.,-8.43374090490393E-31,1.4081690688991E-16));
#125463=DIRECTION('center_axis',(-1.22464679914736E-16,1.,6.98296267768627E-15));
#125464=DIRECTION('ref_axis',(1.,1.22464679914735E-16,1.41265138251802E-16));
#125465=DIRECTION('center_axis',(1.4081690688991E-16,6.98296267768627E-15,
-1.));
#125466=DIRECTION('ref_axis',(-1.,8.42081623376257E-31,-1.40816906889911E-16));
#125467=DIRECTION('center_axis',(-1.4081690688991E-16,-6.98296267768627E-15,
1.));
#125468=DIRECTION('ref_axis',(-1.,1.17957896342593E-30,-1.38342483857788E-16));
#125469=DIRECTION('center_axis',(-1.4081690688991E-16,-6.98296267768627E-15,
1.));
#125470=DIRECTION('ref_axis',(-1.,1.14629496755776E-30,-1.4081690688991E-16));
#125471=DIRECTION('center_axis',(-1.22464679914735E-16,1.,6.98296267768627E-15));
#125472=DIRECTION('ref_axis',(1.,1.22464679914734E-16,1.38342483857788E-16));
#125473=DIRECTION('center_axis',(1.4081690688991E-16,6.98296267768627E-15,
-1.));
#125474=DIRECTION('ref_axis',(-1.,1.19573562666198E-30,-1.40816906889911E-16));
#125475=DIRECTION('center_axis',(1.4081690688991E-16,6.98296267768627E-15,
-1.));
#125476=DIRECTION('ref_axis',(-1.,1.19573562666198E-30,-1.40816906889911E-16));
#125477=DIRECTION('center_axis',(-1.4081690688991E-16,-6.98296267768627E-15,
1.));
#125478=DIRECTION('ref_axis',(-1.,1.17793481601532E-30,-1.38149656210243E-16));
#125479=DIRECTION('center_axis',(-1.4081690688991E-16,-6.98296267768627E-15,
1.));
#125480=DIRECTION('ref_axis',(1.,-1.14470030428736E-30,1.4081690688991E-16));
#125481=DIRECTION('center_axis',(-1.22464679914735E-16,1.,6.98296267768627E-15));
#125482=DIRECTION('ref_axis',(1.,1.22464679914734E-16,1.38149656210243E-16));
#125483=DIRECTION('center_axis',(1.4081690688991E-16,6.98296267768627E-15,
-1.));
#125484=DIRECTION('ref_axis',(-1.,1.14606553893984E-30,-1.40816906889911E-16));
#125485=DIRECTION('center_axis',(-1.4081690688991E-16,-6.98296267768627E-15,
1.));
#125486=DIRECTION('ref_axis',(-1.,1.1860226061992E-30,-1.4081690688991E-16));
#125487=DIRECTION('center_axis',(-1.4081690688991E-16,-6.98296267768627E-15,
1.));
#125488=DIRECTION('ref_axis',(-1.,1.09611010944228E-30,-1.4081690688991E-16));
#125489=DIRECTION('',(1.4081690688991E-16,6.98296267768627E-15,-1.));
#125490=DIRECTION('center_axis',(-1.4081690688991E-16,-6.98296267768627E-15,
1.));
#125491=DIRECTION('ref_axis',(-1.,1.14270052978402E-30,-1.4081690688991E-16));
#125492=DIRECTION('center_axis',(-1.4081690688991E-16,-6.98296267768627E-15,
1.));
#125493=DIRECTION('ref_axis',(-1.,1.14517058122326E-30,-1.4081690688991E-16));
#125494=DIRECTION('',(-0.529919264233199,5.85699181126827E-15,-0.84804809615643));
#125495=DIRECTION('center_axis',(1.4081690688991E-16,6.98296267768627E-15,
-1.));
#125496=DIRECTION('ref_axis',(1.,-8.0229549381324E-31,1.4081690688991E-16));
#125497=DIRECTION('center_axis',(-1.4081690688991E-16,-6.98296267768627E-15,
1.));
#125498=DIRECTION('ref_axis',(1.,-1.19598452005484E-30,1.4081690688991E-16));
#125499=DIRECTION('',(-0.529924202082878,4.64200439806007E-6,0.848045010612807));
#125500=DIRECTION('center_axis',(-1.4081690688991E-16,-6.98296267768627E-15,
1.));
#125501=DIRECTION('ref_axis',(1.,-8.02836526847902E-31,1.4081690688991E-16));
#125502=DIRECTION('',(0.527020736635427,0.0553967790670863,-0.848045010612788));
#125503=DIRECTION('center_axis',(-1.4081690688991E-16,-6.98296267768627E-15,
1.));
#125504=DIRECTION('ref_axis',(1.,-6.21724893790088E-15,1.40816906889867E-16));
#125505=DIRECTION('',(-0.527021707078575,-0.055387545917055,0.848045010612804));
#125506=DIRECTION('center_axis',(-1.4081690688991E-16,-6.98296267768627E-15,
1.));
#125507=DIRECTION('ref_axis',(1.,-8.02836526847902E-31,1.4081690688991E-16));
#125508=DIRECTION('',(0.518343121711171,0.110181977425787,-0.848045010612799));
#125509=DIRECTION('center_axis',(-1.4081690688991E-16,-6.98296267768627E-15,
1.));
#125510=DIRECTION('ref_axis',(1.,-1.24344978758018E-14,1.40816906889824E-16));
#125511=DIRECTION('',(-0.518345051965149,-0.110172896294845,0.848045010612793));
#125512=DIRECTION('center_axis',(-1.4081690688991E-16,-6.98296267768627E-15,
1.));
#125513=DIRECTION('ref_axis',(1.,-8.02836526847902E-31,1.4081690688991E-16));
#125514=DIRECTION('',(0.503986431075191,0.16375999898274,-0.8480450106128));
#125515=DIRECTION('center_axis',(-1.4081690688991E-16,-6.98296267768627E-15,
1.));
#125516=DIRECTION('ref_axis',(1.,-1.19598452005484E-30,1.4081690688991E-16));
#125517=DIRECTION('',(-0.503989299991689,-0.163751169365674,0.848045010612798));
#125518=DIRECTION('center_axis',(-1.4081690688991E-16,-6.98296267768627E-15,
1.));
#125519=DIRECTION('ref_axis',(1.,-8.02836526847902E-31,1.4081690688991E-16));
#125520=DIRECTION('',(0.484107959634417,0.215543831721869,-0.848045010612795));
#125521=DIRECTION('center_axis',(-1.4081690688991E-16,-6.98296267768627E-15,
1.));
#125522=DIRECTION('ref_axis',(1.,-4.79616346638068E-14,1.40816906889576E-16));
#125523=DIRECTION('',(-0.484111735780992,-0.215535350357788,0.848045010612797));
#125524=DIRECTION('center_axis',(-1.4081690688991E-16,-6.98296267768627E-15,
1.));
#125525=DIRECTION('ref_axis',(1.,-8.88178419700127E-16,1.40816906889904E-16));
#125526=DIRECTION('',(0.458925500081787,0.264966121135203,-0.848045010612789));
#125527=DIRECTION('center_axis',(-1.4081690688991E-16,-6.98296267768627E-15,
1.));
#125528=DIRECTION('ref_axis',(1.,-1.19598452005484E-30,1.4081690688991E-16));
#125529=DIRECTION('',(-0.458930142086182,-0.264958080947721,0.848045010612796));
#125530=DIRECTION('center_axis',(-1.4081690688991E-16,-6.98296267768627E-15,
1.));
#125531=DIRECTION('ref_axis',(1.,-8.88178419700127E-16,1.40816906889904E-16));
#125532=DIRECTION('',(0.428714956713912,0.31148538627764,-0.848045010612796));
#125533=DIRECTION('center_axis',(-1.4081690688991E-16,-6.98296267768627E-15,
1.));
#125534=DIRECTION('ref_axis',(1.,-1.19598452005484E-30,1.4081690688991E-16));
#125535=DIRECTION('',(-0.428720413717374,-0.311477875356759,0.848045010612788));
#125536=DIRECTION('center_axis',(-1.4081690688991E-16,-6.98296267768627E-15,
1.));
#125537=DIRECTION('ref_axis',(1.,-8.88178419700127E-16,1.40816906889904E-16));
#125538=DIRECTION('',(0.393807322565913,0.354591952345519,-0.848045010612797));
#125539=DIRECTION('center_axis',(-1.4081690688991E-16,-6.98296267768627E-15,
1.));
#125540=DIRECTION('ref_axis',(1.,-1.19598452005484E-30,1.4081690688991E-16));
#125541=DIRECTION('',(-0.393813534780367,-0.354585052982427,0.848045010612787));
#125542=DIRECTION('center_axis',(-1.4081690688991E-16,-6.98296267768627E-15,
1.));
#125543=DIRECTION('ref_axis',(1.,-8.88178419700127E-16,1.40816906889904E-16));
#125544=DIRECTION('',(0.354585052982402,0.393813534780382,-0.848045010612791));
#125545=DIRECTION('center_axis',(-1.4081690688991E-16,-6.98296267768627E-15,
1.));
#125546=DIRECTION('ref_axis',(1.,-1.19598452005484E-30,1.4081690688991E-16));
#125547=DIRECTION('',(-0.354591952345514,-0.393807322565934,0.84804501061279));
#125548=DIRECTION('center_axis',(-1.4081690688991E-16,-6.98296267768627E-15,
1.));
#125549=DIRECTION('ref_axis',(1.,-8.88178419700127E-16,1.40816906889904E-16));
#125550=DIRECTION('',(0.311477875356731,0.428720413717367,-0.848045010612801));
#125551=DIRECTION('center_axis',(-1.4081690688991E-16,-6.98296267768627E-15,
1.));
#125552=DIRECTION('ref_axis',(1.,-1.19598452005484E-30,1.4081690688991E-16));
#125553=DIRECTION('',(-0.311485386277638,-0.428714956713914,0.848045010612796));
#125554=DIRECTION('center_axis',(-1.4081690688991E-16,-6.98296267768627E-15,
1.));
#125555=DIRECTION('ref_axis',(1.,-8.02836526847902E-31,1.4081690688991E-16));
#125556=DIRECTION('',(0.264958080947702,0.458930142086184,-0.848045010612801));
#125557=DIRECTION('center_axis',(-1.4081690688991E-16,-6.98296267768627E-15,
1.));
#125558=DIRECTION('ref_axis',(1.,-1.19598452005484E-30,1.4081690688991E-16));
#125559=DIRECTION('',(-0.26496612113518,-0.458925500081782,0.8480450106128));
#125560=DIRECTION('center_axis',(-1.4081690688991E-16,-6.98296267768627E-15,
1.));
#125561=DIRECTION('ref_axis',(1.,-8.02836526847902E-31,1.4081690688991E-16));
#125562=DIRECTION('',(0.215535350357773,0.484111735781,-0.848045010612798));
#125563=DIRECTION('center_axis',(-1.4081690688991E-16,-6.98296267768627E-15,
1.));
#125564=DIRECTION('ref_axis',(1.,-1.19598452005484E-30,1.4081690688991E-16));
#125565=DIRECTION('',(-0.215543831721857,-0.484107959634406,0.848045010612805));
#125566=DIRECTION('center_axis',(-1.4081690688991E-16,-6.98296267768627E-15,
1.));
#125567=DIRECTION('ref_axis',(1.,-8.02836526847902E-31,1.4081690688991E-16));
#125568=DIRECTION('',(0.163751169365655,0.503989299991706,-0.848045010612792));
#125569=DIRECTION('center_axis',(-1.4081690688991E-16,-6.98296267768627E-15,
1.));
#125570=DIRECTION('ref_axis',(1.,-1.19598452005484E-30,1.4081690688991E-16));
#125571=DIRECTION('',(-0.163759998982739,-0.5039864310752,0.848045010612796));
#125572=DIRECTION('center_axis',(-1.4081690688991E-16,-6.98296267768627E-15,
1.));
#125573=DIRECTION('ref_axis',(1.,-8.02836526847902E-31,1.4081690688991E-16));
#125574=DIRECTION('',(0.110172896294836,0.518345051965155,-0.848045010612791));
#125575=DIRECTION('center_axis',(-1.4081690688991E-16,-6.98296267768627E-15,
1.));
#125576=DIRECTION('ref_axis',(1.,-1.19598452005484E-30,1.4081690688991E-16));
#125577=DIRECTION('',(-0.110181977425776,-0.518343121711191,0.848045010612788));
#125578=DIRECTION('center_axis',(-1.4081690688991E-16,-6.98296267768627E-15,
1.));
#125579=DIRECTION('ref_axis',(1.,-8.02836526847902E-31,1.4081690688991E-16));
#125580=DIRECTION('',(0.0553875459170424,0.527021707078595,-0.848045010612793));
#125581=DIRECTION('center_axis',(-1.4081690688991E-16,-6.98296267768627E-15,
1.));
#125582=DIRECTION('ref_axis',(1.,-1.19598452005484E-30,1.4081690688991E-16));
#125583=DIRECTION('',(-0.0553967790670788,-0.527020736635434,0.848045010612784));
#125584=DIRECTION('center_axis',(-1.4081690688991E-16,-6.98296267768627E-15,
1.));
#125585=DIRECTION('ref_axis',(1.,-8.02836526847902E-31,1.4081690688991E-16));
#125586=DIRECTION('',(-4.64200440569701E-6,0.529924202082914,-0.848045010612785));
#125587=DIRECTION('center_axis',(-1.4081690688991E-16,-6.98296267768627E-15,
1.));
#125588=DIRECTION('ref_axis',(1.,-1.19598452005484E-30,1.4081690688991E-16));
#125589=DIRECTION('',(-4.64200440229132E-6,-0.529924202082886,0.848045010612803));
#125590=DIRECTION('center_axis',(-1.4081690688991E-16,-6.98296267768627E-15,
1.));
#125591=DIRECTION('ref_axis',(1.,-8.02836526847902E-31,1.4081690688991E-16));
#125592=DIRECTION('',(-0.0553967790670825,0.527020736635425,-0.84804501061279));
#125593=DIRECTION('center_axis',(-1.4081690688991E-16,-6.98296267768627E-15,
1.));
#125594=DIRECTION('ref_axis',(1.,-1.19598452005484E-30,1.4081690688991E-16));
#125595=DIRECTION('',(0.0553875459170465,-0.527021707078599,0.848045010612789));
#125596=DIRECTION('center_axis',(-1.4081690688991E-16,-6.98296267768627E-15,
1.));
#125597=DIRECTION('ref_axis',(1.,-8.02836526847902E-31,1.4081690688991E-16));
#125598=DIRECTION('',(-0.110181977425775,0.518343121711176,-0.848045010612797));
#125599=DIRECTION('center_axis',(-1.4081690688991E-16,-6.98296267768627E-15,
1.));
#125600=DIRECTION('ref_axis',(1.,-1.19598452005484E-30,1.4081690688991E-16));
#125601=DIRECTION('',(0.110172896294839,-0.51834505196514,0.848045010612799));
#125602=DIRECTION('center_axis',(-1.4081690688991E-16,-6.98296267768627E-15,
1.));
#125603=DIRECTION('ref_axis',(1.,-8.02836526847902E-31,1.4081690688991E-16));
#125604=DIRECTION('',(-0.163759998982728,0.50398643107521,-0.848045010612791));
#125605=DIRECTION('center_axis',(-1.4081690688991E-16,-6.98296267768627E-15,
1.));
#125606=DIRECTION('ref_axis',(1.,-1.19598452005484E-30,1.4081690688991E-16));
#125607=DIRECTION('',(0.163751169365666,-0.503989299991696,0.848045010612796));
#125608=DIRECTION('center_axis',(-1.4081690688991E-16,-6.98296267768627E-15,
1.));
#125609=DIRECTION('ref_axis',(1.,-8.02836526847902E-31,1.4081690688991E-16));
#125610=DIRECTION('',(-0.215543831721853,0.484107959634437,-0.848045010612788));
#125611=DIRECTION('center_axis',(-1.4081690688991E-16,-6.98296267768627E-15,
1.));
#125612=DIRECTION('ref_axis',(1.,-1.19598452005484E-30,1.4081690688991E-16));
#125613=DIRECTION('',(0.215535350357773,-0.484111735781,0.848045010612798));
#125614=DIRECTION('center_axis',(-1.4081690688991E-16,-6.98296267768627E-15,
1.));
#125615=DIRECTION('ref_axis',(1.,4.44089209850063E-15,1.40816906889941E-16));
#125616=DIRECTION('',(-0.264966121135185,0.45892550008179,-0.848045010612794));
#125617=DIRECTION('center_axis',(-1.4081690688991E-16,-6.98296267768627E-15,
1.));
#125618=DIRECTION('ref_axis',(1.,-1.19598452005484E-30,1.4081690688991E-16));
#125619=DIRECTION('',(0.264958080947719,-0.458930142086191,0.848045010612792));
#125620=DIRECTION('center_axis',(-1.4081690688991E-16,-6.98296267768627E-15,
1.));
#125621=DIRECTION('ref_axis',(1.,-8.02836526847902E-31,1.4081690688991E-16));
#125622=DIRECTION('',(-0.31148538627764,0.428714956713912,-0.848045010612796));
#125623=DIRECTION('center_axis',(-1.4081690688991E-16,-6.98296267768627E-15,
1.));
#125624=DIRECTION('ref_axis',(1.,-2.01438865587988E-12,1.40816906875844E-16));
#125625=DIRECTION('',(0.31147787535674,-0.428720413717385,0.848045010612789));
#125626=DIRECTION('center_axis',(-1.4081690688991E-16,-6.98296267768627E-15,
1.));
#125627=DIRECTION('ref_axis',(1.,-8.02836526847902E-31,1.4081690688991E-16));
#125628=DIRECTION('',(-0.354591952345504,0.393807322565925,-0.848045010612798));
#125629=DIRECTION('center_axis',(-1.4081690688991E-16,-6.98296267768627E-15,
1.));
#125630=DIRECTION('ref_axis',(1.,-1.19598452005484E-30,1.4081690688991E-16));
#125631=DIRECTION('',(0.354585052982402,-0.393813534780382,0.848045010612791));
#125632=DIRECTION('center_axis',(-1.4081690688991E-16,-6.98296267768627E-15,
1.));
#125633=DIRECTION('ref_axis',(1.,-8.02836526847902E-31,1.4081690688991E-16));
#125634=DIRECTION('',(-0.393813534780341,0.354585052982428,-0.848045010612799));
#125635=DIRECTION('center_axis',(-1.4081690688991E-16,-6.98296267768627E-15,
1.));
#125636=DIRECTION('ref_axis',(1.,2.20534701611541E-12,1.4081690690531E-16));
#125637=DIRECTION('',(0.393807322565921,-0.354591952345514,0.848045010612796));
#125638=DIRECTION('center_axis',(-1.4081690688991E-16,-6.98296267768627E-15,
1.));
#125639=DIRECTION('ref_axis',(1.,-1.24344978758018E-14,1.40816906889824E-16));
#125640=DIRECTION('',(-0.428720413717363,0.311477875356744,-0.848045010612799));
#125641=DIRECTION('center_axis',(-1.4081690688991E-16,-6.98296267768627E-15,
1.));
#125642=DIRECTION('ref_axis',(1.,-1.19598452005484E-30,1.4081690688991E-16));
#125643=DIRECTION('',(0.428714956713901,-0.311485386277647,0.848045010612799));
#125644=DIRECTION('center_axis',(-1.4081690688991E-16,-6.98296267768627E-15,
1.));
#125645=DIRECTION('ref_axis',(1.,-8.02836526847902E-31,1.4081690688991E-16));
#125646=DIRECTION('',(-0.458930142086183,0.264958080947715,-0.848045010612797));
#125647=DIRECTION('center_axis',(-1.4081690688991E-16,-6.98296267768627E-15,
1.));
#125648=DIRECTION('ref_axis',(1.,-1.19598452005484E-30,1.4081690688991E-16));
#125649=DIRECTION('',(0.458925500081769,-0.264966121135201,0.8480450106128));
#125650=DIRECTION('center_axis',(-1.4081690688991E-16,-6.98296267768627E-15,
1.));
#125651=DIRECTION('ref_axis',(1.,-8.02836526847902E-31,1.4081690688991E-16));
#125652=DIRECTION('',(-0.484111735781003,0.215535350357781,-0.848045010612793));
#125653=DIRECTION('center_axis',(-1.4081690688991E-16,-6.98296267768627E-15,
1.));
#125654=DIRECTION('ref_axis',(1.,-1.19598452005484E-30,1.4081690688991E-16));
#125655=DIRECTION('',(0.4841079596344,-0.215543831721854,0.848045010612809));
#125656=DIRECTION('center_axis',(-1.4081690688991E-16,-6.98296267768627E-15,
1.));
#125657=DIRECTION('ref_axis',(1.,-8.02836526847902E-31,1.4081690688991E-16));
#125658=DIRECTION('',(-0.5039892999917,0.163751169365664,-0.848045010612794));
#125659=DIRECTION('center_axis',(-1.4081690688991E-16,-6.98296267768627E-15,
1.));
#125660=DIRECTION('ref_axis',(1.,-1.19598452005484E-30,1.4081690688991E-16));
#125661=DIRECTION('',(0.503986431075195,-0.163759998982748,0.848045010612796));
#125662=DIRECTION('center_axis',(-1.4081690688991E-16,-6.98296267768627E-15,
1.));
#125663=DIRECTION('ref_axis',(1.,-8.02836526847902E-31,1.4081690688991E-16));
#125664=DIRECTION('',(-0.518345051965131,0.11017289629484,-0.848045010612805));
#125665=DIRECTION('center_axis',(-1.4081690688991E-16,-6.98296267768627E-15,
1.));
#125666=DIRECTION('ref_axis',(1.,-1.19598452005484E-30,1.4081690688991E-16));
#125667=DIRECTION('',(0.518343121711172,-0.110181977425781,0.848045010612799));
#125668=DIRECTION('center_axis',(-1.4081690688991E-16,-6.98296267768627E-15,
1.));
#125669=DIRECTION('ref_axis',(1.,-8.02836526847902E-31,1.4081690688991E-16));
#125670=DIRECTION('',(-0.527021707078581,0.0553875459170459,-0.848045010612801));
#125671=DIRECTION('center_axis',(-1.4081690688991E-16,-6.98296267768627E-15,
1.));
#125672=DIRECTION('ref_axis',(1.,-1.19598452005484E-30,1.4081690688991E-16));
#125673=DIRECTION('',(0.527020736635404,-0.0553967790670833,0.848045010612803));
#125674=DIRECTION('center_axis',(-1.4081690688991E-16,-6.98296267768627E-15,
1.));
#125675=DIRECTION('ref_axis',(1.,-8.02836526847902E-31,1.4081690688991E-16));
#125676=DIRECTION('',(-0.529924202082893,-4.64200439816316E-6,-0.848045010612798));
#125677=DIRECTION('',(-0.529919264233196,5.98678459741823E-15,-0.848048096156432));
#125678=DIRECTION('',(0.529924202082893,-4.64200440982505E-6,0.848045010612798));
#125679=DIRECTION('center_axis',(-1.4081690688991E-16,-6.98296267768627E-15,
1.));
#125680=DIRECTION('ref_axis',(1.,-8.02836526847902E-31,1.4081690688991E-16));
#125681=DIRECTION('',(-0.527020736635413,-0.0553967790670796,-0.848045010612797));
#125682=DIRECTION('center_axis',(-1.4081690688991E-16,-6.98296267768627E-15,
1.));
#125683=DIRECTION('ref_axis',(1.,-1.19598452005484E-30,1.4081690688991E-16));
#125684=DIRECTION('',(0.527021707078571,0.0553875459170413,0.848045010612807));
#125685=DIRECTION('center_axis',(-1.4081690688991E-16,-6.98296267768627E-15,
1.));
#125686=DIRECTION('ref_axis',(1.,-8.02836526847902E-31,1.4081690688991E-16));
#125687=DIRECTION('',(-0.518343121711153,-0.110181977425773,-0.848045010612811));
#125688=DIRECTION('center_axis',(-1.4081690688991E-16,-6.98296267768627E-15,
1.));
#125689=DIRECTION('ref_axis',(1.,-1.19598452005484E-30,1.4081690688991E-16));
#125690=DIRECTION('',(0.518345051965141,0.110172896294833,0.848045010612799));
#125691=DIRECTION('center_axis',(-1.4081690688991E-16,-6.98296267768627E-15,
1.));
#125692=DIRECTION('ref_axis',(1.,-8.02836526847902E-31,1.4081690688991E-16));
#125693=DIRECTION('',(-0.503986431075192,-0.163759998982734,-0.848045010612801));
#125694=DIRECTION('center_axis',(-1.4081690688991E-16,-6.98296267768627E-15,
1.));
#125695=DIRECTION('ref_axis',(1.,-1.19598452005484E-30,1.4081690688991E-16));
#125696=DIRECTION('',(0.503989299991687,0.163751169365657,0.848045010612803));
#125697=DIRECTION('center_axis',(-1.4081690688991E-16,-6.98296267768627E-15,
1.));
#125698=DIRECTION('ref_axis',(1.,-8.02836526847902E-31,1.4081690688991E-16));
#125699=DIRECTION('',(-0.484107959634419,-0.21554383172185,-0.848045010612799));
#125700=DIRECTION('center_axis',(-1.4081690688991E-16,-6.98296267768627E-15,
1.));
#125701=DIRECTION('ref_axis',(1.,-1.19598452005484E-30,1.4081690688991E-16));
#125702=DIRECTION('',(0.484111735780995,0.21553535035777,0.848045010612801));
#125703=DIRECTION('center_axis',(-1.4081690688991E-16,-6.98296267768627E-15,
1.));
#125704=DIRECTION('ref_axis',(1.,-8.02836526847902E-31,1.4081690688991E-16));
#125705=DIRECTION('',(-0.458925500081788,-0.264966121135171,-0.8480450106128));
#125706=DIRECTION('center_axis',(-1.4081690688991E-16,-6.98296267768627E-15,
1.));
#125707=DIRECTION('ref_axis',(1.,-1.19598452005484E-30,1.4081690688991E-16));
#125708=DIRECTION('',(0.45893014208618,0.264958080947707,0.848045010612802));
#125709=DIRECTION('center_axis',(-1.4081690688991E-16,-6.98296267768627E-15,
1.));
#125710=DIRECTION('ref_axis',(1.,-8.02836526847902E-31,1.4081690688991E-16));
#125711=DIRECTION('',(-0.428714956713899,-0.311485386277633,-0.848045010612806));
#125712=DIRECTION('center_axis',(-1.4081690688991E-16,-6.98296267768627E-15,
1.));
#125713=DIRECTION('ref_axis',(1.,-1.19598452005484E-30,1.4081690688991E-16));
#125714=DIRECTION('',(0.42872041371736,0.311477875356735,0.848045010612803));
#125715=DIRECTION('center_axis',(-1.4081690688991E-16,-6.98296267768627E-15,
1.));
#125716=DIRECTION('ref_axis',(1.,-8.02836526847902E-31,1.4081690688991E-16));
#125717=DIRECTION('',(-0.393807322565921,-0.354591952345514,-0.848045010612796));
#125718=DIRECTION('center_axis',(-1.4081690688991E-16,-6.98296267768627E-15,
1.));
#125719=DIRECTION('ref_axis',(1.,-1.19598452005484E-30,1.4081690688991E-16));
#125720=DIRECTION('',(0.393813534780356,0.354585052982402,0.848045010612803));
#125721=DIRECTION('center_axis',(-1.4081690688991E-16,-6.98296267768627E-15,
1.));
#125722=DIRECTION('ref_axis',(1.,-8.02836526847902E-31,1.4081690688991E-16));
#125723=DIRECTION('',(-0.354585052982407,-0.393813534780348,-0.848045010612804));
#125724=DIRECTION('center_axis',(-1.4081690688991E-16,-6.98296267768627E-15,
1.));
#125725=DIRECTION('ref_axis',(1.,-1.19598452005484E-30,1.4081690688991E-16));
#125726=DIRECTION('',(0.354591952345508,0.393807322565902,0.848045010612807));
#125727=DIRECTION('center_axis',(-1.4081690688991E-16,-6.98296267768627E-15,
1.));
#125728=DIRECTION('ref_axis',(1.,-8.02836526847902E-31,1.4081690688991E-16));
#125729=DIRECTION('',(-0.311477875356729,-0.428720413717378,-0.848045010612797));
#125730=DIRECTION('center_axis',(-1.4081690688991E-16,-6.98296267768627E-15,
1.));
#125731=DIRECTION('ref_axis',(1.,-7.47846229387506E-12,1.40816906837689E-16));
#125732=DIRECTION('',(0.311485386277628,0.428714956713906,0.848045010612804));
#125733=DIRECTION('center_axis',(-1.4081690688991E-16,-6.98296267768627E-15,
1.));
#125734=DIRECTION('ref_axis',(1.,1.95399252334028E-14,1.40816906890047E-16));
#125735=DIRECTION('',(-0.264958080947707,-0.458930142086193,-0.848045010612795));
#125736=DIRECTION('center_axis',(-1.4081690688991E-16,-6.98296267768627E-15,
1.));
#125737=DIRECTION('ref_axis',(1.,-7.67208518936968E-12,1.40816906836337E-16));
#125738=DIRECTION('',(0.264966121135178,0.458925500081776,0.848045010612803));
#125739=DIRECTION('center_axis',(-1.4081690688991E-16,-6.98296267768627E-15,
1.));
#125740=DIRECTION('ref_axis',(1.,3.01980662698043E-14,1.40816906890121E-16));
#125741=DIRECTION('',(-0.215535350357775,-0.484111735780979,-0.848045010612808));
#125742=DIRECTION('center_axis',(-1.4081690688991E-16,-6.98296267768627E-15,
1.));
#125743=DIRECTION('ref_axis',(1.,5.89750470680883E-12,1.40816906931093E-16));
#125744=DIRECTION('',(0.21554383172186,0.484107959634412,0.848045010612801));
#125745=DIRECTION('center_axis',(-1.4081690688991E-16,-6.98296267768627E-15,
1.));
#125746=DIRECTION('ref_axis',(1.,-8.02836526847902E-31,1.4081690688991E-16));
#125747=DIRECTION('',(-0.163751169365654,-0.503989299991677,-0.848045010612809));
#125748=DIRECTION('center_axis',(-1.4081690688991E-16,-6.98296267768627E-15,
1.));
#125749=DIRECTION('ref_axis',(1.,6.04050143238055E-12,1.40816906932091E-16));
#125750=DIRECTION('',(0.163759998982731,0.503986431075181,0.848045010612808));
#125751=DIRECTION('center_axis',(-1.4081690688991E-16,-6.98296267768627E-15,
1.));
#125752=DIRECTION('ref_axis',(1.,-2.1316282072803E-14,1.40816906889762E-16));
#125753=DIRECTION('',(-0.110172896294832,-0.51834505196514,-0.8480450106128));
#125754=DIRECTION('center_axis',(-1.4081690688991E-16,-6.98296267768627E-15,
1.));
#125755=DIRECTION('ref_axis',(1.,6.18438633637197E-12,1.40816906933096E-16));
#125756=DIRECTION('',(0.11018197742577,0.518343121711167,0.848045010612803));
#125757=DIRECTION('center_axis',(-1.4081690688991E-16,-6.98296267768627E-15,
1.));
#125758=DIRECTION('ref_axis',(1.,-8.02836526847902E-31,1.4081690688991E-16));
#125759=DIRECTION('',(-0.0553875459170386,-0.52702170707859,-0.848045010612796));
#125760=DIRECTION('center_axis',(-1.4081690688991E-16,-6.98296267768627E-15,
1.));
#125761=DIRECTION('ref_axis',(1.,-2.1094237467878E-12,1.4081690687518E-16));
#125762=DIRECTION('',(0.0553967790670769,0.527020736635406,0.848045010612802));
#125763=DIRECTION('center_axis',(-1.4081690688991E-16,-6.98296267768627E-15,
1.));
#125764=DIRECTION('ref_axis',(1.,-8.02836526847902E-31,1.4081690688991E-16));
#125765=DIRECTION('',(4.64200440982511E-6,-0.5299242020829,-0.848045010612794));
#125766=DIRECTION('',(4.64200439836955E-6,0.52992420208289,0.8480450106128));
#125767=DIRECTION('center_axis',(-1.4081690688991E-16,-6.98296267768627E-15,
1.));
#125768=DIRECTION('ref_axis',(1.,3.37507799486048E-14,1.40816906890146E-16));
#125769=DIRECTION('',(0.0553967790670857,-0.527020736635411,-0.848045010612798));
#125770=DIRECTION('center_axis',(-1.4081690688991E-16,-6.98296267768627E-15,
1.));
#125771=DIRECTION('ref_axis',(1.,-1.19598452005484E-30,1.4081690688991E-16));
#125772=DIRECTION('',(-0.0553875459170506,0.52702170707858,0.848045010612801));
#125773=DIRECTION('center_axis',(-1.4081690688991E-16,-6.98296267768627E-15,
1.));
#125774=DIRECTION('ref_axis',(1.,-1.06581410364015E-14,1.40816906889836E-16));
#125775=DIRECTION('',(0.110181977425778,-0.518343121711171,-0.848045010612799));
#125776=DIRECTION('center_axis',(-1.4081690688991E-16,-6.98296267768627E-15,
1.));
#125777=DIRECTION('ref_axis',(1.,-1.19598452005484E-30,1.4081690688991E-16));
#125778=DIRECTION('',(-0.110172896294836,0.518345051965145,0.848045010612797));
#125779=DIRECTION('center_axis',(-1.4081690688991E-16,-6.98296267768627E-15,
1.));
#125780=DIRECTION('ref_axis',(1.,-1.24344978758018E-14,1.40816906889824E-16));
#125781=DIRECTION('',(0.163759998982748,-0.503986431075193,-0.848045010612797));
#125782=DIRECTION('center_axis',(-1.4081690688991E-16,-6.98296267768627E-15,
1.));
#125783=DIRECTION('ref_axis',(1.,-1.19598452005484E-30,1.4081690688991E-16));
#125784=DIRECTION('',(-0.163751169365665,0.503989299991695,0.848045010612797));
#125785=DIRECTION('center_axis',(-1.4081690688991E-16,-6.98296267768627E-15,
1.));
#125786=DIRECTION('ref_axis',(1.,3.5527136788005E-14,1.40816906890159E-16));
#125787=DIRECTION('',(0.215543831721856,-0.484107959634392,-0.848045010612813));
#125788=DIRECTION('center_axis',(-1.4081690688991E-16,-6.98296267768627E-15,
1.));
#125789=DIRECTION('ref_axis',(1.,-4.69846384021366E-12,1.40816906857101E-16));
#125790=DIRECTION('',(-0.215535350357786,0.484111735780988,0.848045010612801));
#125791=DIRECTION('center_axis',(-1.4081690688991E-16,-6.98296267768627E-15,
1.));
#125792=DIRECTION('ref_axis',(1.,3.5527136788005E-14,1.40816906890159E-16));
#125793=DIRECTION('',(0.264966121135192,-0.458925500081766,-0.848045010612805));
#125794=DIRECTION('center_axis',(-1.4081690688991E-16,-6.98296267768627E-15,
1.));
#125795=DIRECTION('ref_axis',(1.,-2.39719355477064E-12,1.40816906873171E-16));
#125796=DIRECTION('',(-0.264958080947705,0.458930142086164,0.848045010612811));
#125797=DIRECTION('center_axis',(-1.4081690688991E-16,-6.98296267768627E-15,
1.));
#125798=DIRECTION('ref_axis',(1.,4.2632564145606E-14,1.40816906890208E-16));
#125799=DIRECTION('',(0.311485386277635,-0.428714956713879,-0.848045010612815));
#125800=DIRECTION('center_axis',(-1.4081690688991E-16,-6.98296267768627E-15,
1.));
#125801=DIRECTION('ref_axis',(1.,-1.22213350550737E-12,1.40816906881376E-16));
#125802=DIRECTION('',(-0.311477875356741,0.428720413717359,0.848045010612802));
#125803=DIRECTION('center_axis',(-1.4081690688991E-16,-6.98296267768627E-15,
1.));
#125804=DIRECTION('ref_axis',(1.,3.10862446895044E-14,1.40816906890128E-16));
#125805=DIRECTION('',(0.354591952345524,-0.393807322565893,-0.848045010612805));
#125806=DIRECTION('center_axis',(-1.4081690688991E-16,-6.98296267768627E-15,
1.));
#125807=DIRECTION('ref_axis',(1.,4.9862336481965E-12,1.40816906924729E-16));
#125808=DIRECTION('',(-0.354585052982407,0.393813534780348,0.848045010612804));
#125809=DIRECTION('center_axis',(-1.4081690688991E-16,-6.98296267768627E-15,
1.));
#125810=DIRECTION('ref_axis',(1.,-8.02836526847902E-31,1.4081690688991E-16));
#125811=DIRECTION('',(0.393813534780361,-0.354585052982394,-0.848045010612804));
#125812=DIRECTION('center_axis',(-1.4081690688991E-16,-6.98296267768627E-15,
1.));
#125813=DIRECTION('ref_axis',(1.,-1.27009514017118E-12,1.40816906881041E-16));
#125814=DIRECTION('',(-0.393807322565913,0.354591952345492,0.848045010612809));
#125815=DIRECTION('center_axis',(-1.4081690688991E-16,-6.98296267768627E-15,
1.));
#125816=DIRECTION('ref_axis',(1.,3.90798504668055E-14,1.40816906890183E-16));
#125817=DIRECTION('',(0.428720413717362,-0.311477875356717,-0.848045010612809));
#125818=DIRECTION('center_axis',(-1.4081690688991E-16,-6.98296267768627E-15,
1.));
#125819=DIRECTION('ref_axis',(1.,-2.58904009342587E-12,1.40816906871831E-16));
#125820=DIRECTION('',(-0.428714956713912,0.311485386277613,0.848045010612806));
#125821=DIRECTION('center_axis',(-1.4081690688991E-16,-6.98296267768627E-15,
1.));
#125822=DIRECTION('ref_axis',(1.,3.99680288865056E-14,1.4081690689019E-16));
#125823=DIRECTION('',(0.458930142086181,-0.264958080947701,-0.848045010612803));
#125824=DIRECTION('center_axis',(-1.4081690688991E-16,-6.98296267768627E-15,
1.));
#125825=DIRECTION('ref_axis',(1.,-1.19598452005484E-30,1.4081690688991E-16));
#125826=DIRECTION('',(-0.458925500081773,0.26496612113517,0.848045010612808));
#125827=DIRECTION('center_axis',(-1.4081690688991E-16,-6.98296267768627E-15,
1.));
#125828=DIRECTION('ref_axis',(1.,-9.76996261670138E-15,1.40816906889842E-16));
#125829=DIRECTION('',(0.484111735780991,-0.215535350357761,-0.848045010612805));
#125830=DIRECTION('center_axis',(-1.4081690688991E-16,-6.98296267768627E-15,
1.));
#125831=DIRECTION('ref_axis',(1.,-2.01350047746018E-12,1.4081690687585E-16));
#125832=DIRECTION('',(-0.484107959634416,0.215543831721835,0.848045010612804));
#125833=DIRECTION('center_axis',(-1.4081690688991E-16,-6.98296267768627E-15,
1.));
#125834=DIRECTION('ref_axis',(1.,-1.4210854715202E-14,1.40816906889811E-16));
#125835=DIRECTION('',(0.503989299991706,-0.163751169365648,-0.848045010612793));
#125836=DIRECTION('center_axis',(-1.4081690688991E-16,-6.98296267768627E-15,
1.));
#125837=DIRECTION('ref_axis',(1.,-1.36601840949879E-12,1.40816906880372E-16));
#125838=DIRECTION('',(-0.503986431075204,0.16375999898272,0.848045010612797));
#125839=DIRECTION('center_axis',(-1.4081690688991E-16,-6.98296267768627E-15,
1.));
#125840=DIRECTION('ref_axis',(1.,-1.24344978758018E-14,1.40816906889824E-16));
#125841=DIRECTION('',(0.518345051965146,-0.110172896294824,-0.848045010612797));
#125842=DIRECTION('center_axis',(-1.4081690688991E-16,-6.98296267768627E-15,
1.));
#125843=DIRECTION('ref_axis',(1.,-2.78088663208109E-12,1.40816906870492E-16));
#125844=DIRECTION('',(-0.518343121711178,0.110181977425763,0.848045010612798));
#125845=DIRECTION('center_axis',(-1.4081690688991E-16,-6.98296267768627E-15,
1.));
#125846=DIRECTION('ref_axis',(1.,-1.59872115546023E-14,1.40816906889799E-16));
#125847=DIRECTION('',(0.527021707078576,-0.0553875459170319,-0.848045010612805));
#125848=DIRECTION('center_axis',(-1.4081690688991E-16,-6.98296267768627E-15,
1.));
#125849=DIRECTION('ref_axis',(1.,-2.65121258280487E-12,1.40816906871397E-16));
#125850=DIRECTION('',(-0.527020736635418,0.0553967790670702,0.848045010612795));
#125851=DIRECTION('center_axis',(-1.4081690688991E-16,-6.98296267768627E-15,
1.));
#125852=DIRECTION('ref_axis',(1.,-2.75335310107039E-14,1.40816906889718E-16));
#125853=DIRECTION('',(0.529924202082878,4.64200440992836E-6,-0.848045010612807));
#125854=DIRECTION('center_axis',(-1.4081690688991E-16,-6.98296267768627E-15,
1.));
#125855=DIRECTION('ref_axis',(-1.,8.42929103913772E-31,-1.4081690688991E-16));
#125856=DIRECTION('',(-0.529924689637705,5.13655125493133E-6,0.848044705947746));
#125857=DIRECTION('center_axis',(1.4081690688991E-16,6.98296267768627E-15,
-1.));
#125858=DIRECTION('ref_axis',(-1.,8.44830660832796E-31,-1.4081690688991E-16));
#125859=DIRECTION('',(0.527022243656736,-0.0553871050427146,-0.848044705947751));
#125860=DIRECTION('center_axis',(1.4081690688991E-16,6.98296267768627E-15,
-1.));
#125861=DIRECTION('ref_axis',(-1.,8.43549292198398E-31,-1.4081690688991E-16));
#125862=DIRECTION('',(-0.527021169825118,0.0553973218681055,0.84804470594775));
#125863=DIRECTION('center_axis',(1.4081690688991E-16,6.98296267768627E-15,
-1.));
#125864=DIRECTION('ref_axis',(-1.,8.44830660832796E-31,-1.4081690688991E-16));
#125865=DIRECTION('',(0.518345631687772,-0.110172513923351,-0.848044705947755));
#125866=DIRECTION('center_axis',(1.4081690688991E-16,6.98296267768627E-15,
-1.));
#125867=DIRECTION('ref_axis',(-1.,1.06581410364015E-14,-1.40816906889836E-16));
#125868=DIRECTION('',(-0.51834349578966,0.110182562533931,0.848044705947753));
#125869=DIRECTION('center_axis',(1.4081690688991E-16,6.98296267768627E-15,
-1.));
#125870=DIRECTION('ref_axis',(-1.,8.44830660832796E-31,-1.4081690688991E-16));
#125871=DIRECTION('',(0.50398991650726,-0.163750849686354,-0.848044705947748));
#125872=DIRECTION('center_axis',(1.4081690688991E-16,6.98296267768627E-15,
-1.));
#125873=DIRECTION('ref_axis',(-1.,3.37507799486048E-14,-1.40816906889675E-16));
#125874=DIRECTION('',(-0.50398674194399,0.163760619987459,0.848044705947749));
#125875=DIRECTION('center_axis',(1.4081690688991E-16,6.98296267768627E-15,
-1.));
#125876=DIRECTION('ref_axis',(-1.,8.44830660832796E-31,-1.4081690688991E-16));
#125877=DIRECTION('',(0.484112382334808,-0.215535096873135,-0.848044705947749));
#125878=DIRECTION('center_axis',(1.4081690688991E-16,6.98296267768627E-15,
-1.));
#125879=DIRECTION('ref_axis',(-1.,-4.52970994047064E-14,-1.40816906890227E-16));
#125880=DIRECTION('',(-0.484108203887568,0.215544481819274,0.848044705947754));
#125881=DIRECTION('center_axis',(1.4081690688991E-16,6.98296267768627E-15,
-1.));
#125882=DIRECTION('ref_axis',(-1.,-8.88178419700124E-16,-1.40816906889917E-16));
#125883=DIRECTION('',(0.458930811594458,-0.264957896434951,-0.848044705947757));
#125884=DIRECTION('center_axis',(1.4081690688991E-16,6.98296267768627E-15,
-1.));
#125885=DIRECTION('ref_axis',(-1.,8.43549292198398E-31,-1.4081690688991E-16));
#125886=DIRECTION('',(-0.458925675043199,0.264966793202718,0.848044705947754));
#125887=DIRECTION('center_axis',(1.4081690688991E-16,6.98296267768627E-15,
-1.));
#125888=DIRECTION('ref_axis',(-1.,-8.88178419700124E-16,-1.40816906889917E-16));
#125889=DIRECTION('',(0.428721098844841,-0.311477761837424,-0.848044705947759));
#125890=DIRECTION('center_axis',(1.4081690688991E-16,6.98296267768627E-15,
-1.));
#125891=DIRECTION('ref_axis',(-1.,-1.35003119794419E-13,-1.40816906890853E-16));
#125892=DIRECTION('',(-0.428715060466688,0.311486072951948,0.848044705947757));
#125893=DIRECTION('center_axis',(1.4081690688991E-16,6.98296267768627E-15,
-1.));
#125894=DIRECTION('ref_axis',(-1.,8.44830660832796E-31,-1.4081690688991E-16));
#125895=DIRECTION('',(0.393814228020628,-0.354585011700303,-0.848044705947754));
#125896=DIRECTION('center_axis',(1.4081690688991E-16,6.98296267768627E-15,
-1.));
#125897=DIRECTION('ref_axis',(-1.,-1.58095758706622E-13,-1.40816906891014E-16));
#125898=DIRECTION('',(-0.393807353973301,0.354592646103292,0.848044705947754));
#125899=DIRECTION('center_axis',(1.4081690688991E-16,6.98296267768627E-15,
-1.));
#125900=DIRECTION('ref_axis',(-1.,8.44830660832796E-31,-1.4081690688991E-16));
#125901=DIRECTION('',(0.354592646103302,-0.393807353973285,-0.848044705947757));
#125902=DIRECTION('center_axis',(1.4081690688991E-16,6.98296267768627E-15,
-1.));
#125903=DIRECTION('ref_axis',(-1.,8.43549292198398E-31,-1.4081690688991E-16));
#125904=DIRECTION('',(-0.354585011700314,0.393814228020627,0.84804470594775));
#125905=DIRECTION('center_axis',(1.4081690688991E-16,6.98296267768627E-15,
-1.));
#125906=DIRECTION('ref_axis',(-1.,8.44830660832796E-31,-1.4081690688991E-16));
#125907=DIRECTION('',(0.311486072951975,-0.428715060466675,-0.848044705947754));
#125908=DIRECTION('center_axis',(1.4081690688991E-16,6.98296267768627E-15,
-1.));
#125909=DIRECTION('ref_axis',(-1.,8.43549292198398E-31,-1.4081690688991E-16));
#125910=DIRECTION('',(-0.311477761837451,0.428721098844829,0.848044705947755));
#125911=DIRECTION('center_axis',(1.4081690688991E-16,6.98296267768627E-15,
-1.));
#125912=DIRECTION('ref_axis',(-1.,8.44830660832796E-31,-1.4081690688991E-16));
#125913=DIRECTION('',(0.264966793202735,-0.458925675043194,-0.848044705947751));
#125914=DIRECTION('center_axis',(1.4081690688991E-16,6.98296267768627E-15,
-1.));
#125915=DIRECTION('ref_axis',(-1.,8.43549292198398E-31,-1.4081690688991E-16));
#125916=DIRECTION('',(-0.264957896434977,0.458930811594459,0.848044705947748));
#125917=DIRECTION('center_axis',(1.4081690688991E-16,6.98296267768627E-15,
-1.));
#125918=DIRECTION('ref_axis',(-1.,8.44830660832796E-31,-1.4081690688991E-16));
#125919=DIRECTION('',(0.215544481819299,-0.484108203887551,-0.848044705947758));
#125920=DIRECTION('center_axis',(1.4081690688991E-16,6.98296267768627E-15,
-1.));
#125921=DIRECTION('ref_axis',(-1.,8.43549292198398E-31,-1.4081690688991E-16));
#125922=DIRECTION('',(-0.215535096873164,0.484112382334786,0.848044705947755));
#125923=DIRECTION('center_axis',(1.4081690688991E-16,6.98296267768627E-15,
-1.));
#125924=DIRECTION('ref_axis',(-1.,8.44830660832796E-31,-1.4081690688991E-16));
#125925=DIRECTION('',(0.163760619987462,-0.503986741943988,-0.84804470594775));
#125926=DIRECTION('center_axis',(1.4081690688991E-16,6.98296267768627E-15,
-1.));
#125927=DIRECTION('ref_axis',(-1.,8.43549292198398E-31,-1.4081690688991E-16));
#125928=DIRECTION('',(-0.163750849686384,0.503989916507238,0.848044705947755));
#125929=DIRECTION('center_axis',(1.4081690688991E-16,6.98296267768627E-15,
-1.));
#125930=DIRECTION('ref_axis',(-1.,8.44830660832796E-31,-1.4081690688991E-16));
#125931=DIRECTION('',(0.110182562533939,-0.518343495789657,-0.848044705947754));
#125932=DIRECTION('center_axis',(1.4081690688991E-16,6.98296267768627E-15,
-1.));
#125933=DIRECTION('ref_axis',(-1.,8.43549292198398E-31,-1.4081690688991E-16));
#125934=DIRECTION('',(-0.110172513923364,0.518345631687762,0.848044705947759));
#125935=DIRECTION('center_axis',(1.4081690688991E-16,6.98296267768627E-15,
-1.));
#125936=DIRECTION('ref_axis',(-1.,8.44830660832796E-31,-1.4081690688991E-16));
#125937=DIRECTION('',(0.0553973218681131,-0.527021169825101,-0.84804470594776));
#125938=DIRECTION('center_axis',(1.4081690688991E-16,6.98296267768627E-15,
-1.));
#125939=DIRECTION('ref_axis',(-1.,8.43549292198398E-31,-1.4081690688991E-16));
#125940=DIRECTION('',(-0.0553871050427231,0.527022243656726,0.848044705947757));
#125941=DIRECTION('center_axis',(1.4081690688991E-16,6.98296267768627E-15,
-1.));
#125942=DIRECTION('ref_axis',(-1.,8.44830660832796E-31,-1.4081690688991E-16));
#125943=DIRECTION('',(5.13655126277485E-6,-0.529924689637692,-0.848044705947753));
#125944=DIRECTION('center_axis',(1.4081690688991E-16,6.98296267768627E-15,
-1.));
#125945=DIRECTION('ref_axis',(-1.,8.43549292198398E-31,-1.4081690688991E-16));
#125946=DIRECTION('',(5.13655125885311E-6,0.529924689637688,0.848044705947756));
#125947=DIRECTION('center_axis',(1.4081690688991E-16,6.98296267768627E-15,
-1.));
#125948=DIRECTION('ref_axis',(-1.,8.44830660832796E-31,-1.4081690688991E-16));
#125949=DIRECTION('',(-0.0553871050427198,-0.527022243656726,-0.848044705947757));
#125950=DIRECTION('center_axis',(1.4081690688991E-16,6.98296267768627E-15,
-1.));
#125951=DIRECTION('ref_axis',(-1.,8.43549292198398E-31,-1.4081690688991E-16));
#125952=DIRECTION('',(0.0553973218681098,0.527021169825101,0.84804470594776));
#125953=DIRECTION('center_axis',(1.4081690688991E-16,6.98296267768627E-15,
-1.));
#125954=DIRECTION('ref_axis',(-1.,8.44830660832796E-31,-1.4081690688991E-16));
#125955=DIRECTION('',(-0.110172513923356,-0.518345631687777,-0.848044705947751));
#125956=DIRECTION('center_axis',(1.4081690688991E-16,6.98296267768627E-15,
-1.));
#125957=DIRECTION('ref_axis',(-1.,8.43549292198398E-31,-1.4081690688991E-16));
#125958=DIRECTION('',(0.110182562533938,0.518343495789653,0.848044705947757));
#125959=DIRECTION('center_axis',(1.4081690688991E-16,6.98296267768627E-15,
-1.));
#125960=DIRECTION('ref_axis',(-1.,8.44830660832796E-31,-1.4081690688991E-16));
#125961=DIRECTION('',(-0.163750849686368,-0.503989916507249,-0.848044705947751));
#125962=DIRECTION('center_axis',(1.4081690688991E-16,6.98296267768627E-15,
-1.));
#125963=DIRECTION('ref_axis',(-1.,8.43549292198398E-31,-1.4081690688991E-16));
#125964=DIRECTION('',(0.163760619987469,0.503986741943977,0.848044705947755));
#125965=DIRECTION('center_axis',(1.4081690688991E-16,6.98296267768627E-15,
-1.));
#125966=DIRECTION('ref_axis',(-1.,8.44830660832796E-31,-1.4081690688991E-16));
#125967=DIRECTION('',(-0.215535096873149,-0.484112382334797,-0.848044705947752));
#125968=DIRECTION('center_axis',(1.4081690688991E-16,6.98296267768627E-15,
-1.));
#125969=DIRECTION('ref_axis',(-1.,8.43549292198398E-31,-1.4081690688991E-16));
#125970=DIRECTION('',(0.215544481819295,0.484108203887571,0.848044705947748));
#125971=DIRECTION('center_axis',(1.4081690688991E-16,6.98296267768627E-15,
-1.));
#125972=DIRECTION('ref_axis',(-1.,-5.32907051820075E-15,-1.40816906889948E-16));
#125973=DIRECTION('',(-0.264957896434958,-0.458930811594447,-0.848044705947761));
#125974=DIRECTION('center_axis',(1.4081690688991E-16,6.98296267768627E-15,
-1.));
#125975=DIRECTION('ref_axis',(-1.,-1.80122583515185E-12,-1.40816906902488E-16));
#125976=DIRECTION('',(0.264966793202733,0.45892567504319,0.848044705947754));
#125977=DIRECTION('center_axis',(1.4081690688991E-16,6.98296267768627E-15,
-1.));
#125978=DIRECTION('ref_axis',(-1.,-1.06581410364015E-14,-1.40816906889985E-16));
#125979=DIRECTION('',(-0.311477761837441,-0.428721098844834,-0.848044705947756));
#125980=DIRECTION('center_axis',(1.4081690688991E-16,6.98296267768627E-15,
-1.));
#125981=DIRECTION('ref_axis',(-1.,1.89182003396127E-12,-1.408169068767E-16));
#125982=DIRECTION('',(0.311486072951956,0.42871506046668,0.848044705947758));
#125983=DIRECTION('center_axis',(1.4081690688991E-16,6.98296267768627E-15,
-1.));
#125984=DIRECTION('ref_axis',(-1.,8.44830660832796E-31,-1.4081690688991E-16));
#125985=DIRECTION('',(-0.354585011700305,-0.393814228020624,-0.848044705947755));
#125986=DIRECTION('center_axis',(1.4081690688991E-16,6.98296267768627E-15,
-1.));
#125987=DIRECTION('ref_axis',(-1.,8.43549292198398E-31,-1.4081690688991E-16));
#125988=DIRECTION('',(0.354592646103294,0.39380735397329,0.848044705947758));
#125989=DIRECTION('center_axis',(1.4081690688991E-16,6.98296267768627E-15,
-1.));
#125990=DIRECTION('ref_axis',(-1.,8.44830660832796E-31,-1.4081690688991E-16));
#125991=DIRECTION('',(-0.393807353973315,-0.354592646103273,-0.848044705947756));
#125992=DIRECTION('center_axis',(1.4081690688991E-16,6.98296267768627E-15,
-1.));
#125993=DIRECTION('ref_axis',(-1.,8.43549292198398E-31,-1.4081690688991E-16));
#125994=DIRECTION('',(0.393814228020631,0.354585011700291,0.848044705947758));
#125995=DIRECTION('center_axis',(1.4081690688991E-16,6.98296267768627E-15,
-1.));
#125996=DIRECTION('ref_axis',(-1.,8.44830660832796E-31,-1.4081690688991E-16));
#125997=DIRECTION('',(-0.428715060466688,-0.311486072951948,-0.848044705947757));
#125998=DIRECTION('center_axis',(1.4081690688991E-16,6.98296267768627E-15,
-1.));
#125999=DIRECTION('ref_axis',(-1.,-2.1618262735501E-12,-1.40816906905006E-16));
#126000=DIRECTION('',(0.428721098844841,0.311477761837424,0.848044705947759));
#126001=DIRECTION('center_axis',(1.4081690688991E-16,6.98296267768627E-15,
-1.));
#126002=DIRECTION('ref_axis',(-1.,8.44830660832796E-31,-1.4081690688991E-16));
#126003=DIRECTION('',(-0.458925675043199,-0.264966793202717,-0.848044705947754));
#126004=DIRECTION('center_axis',(1.4081690688991E-16,6.98296267768627E-15,
-1.));
#126005=DIRECTION('ref_axis',(-1.,2.25064411552012E-12,-1.40816906874194E-16));
#126006=DIRECTION('',(0.458930811594462,0.264957896434966,0.84804470594775));
#126007=DIRECTION('center_axis',(1.4081690688991E-16,6.98296267768627E-15,
-1.));
#126008=DIRECTION('ref_axis',(-1.,8.44830660832796E-31,-1.4081690688991E-16));
#126009=DIRECTION('',(-0.484108203887567,-0.215544481819293,-0.84804470594775));
#126010=DIRECTION('center_axis',(1.4081690688991E-16,6.98296267768627E-15,
-1.));
#126011=DIRECTION('ref_axis',(-1.,2.34123831432953E-12,-1.40816906873562E-16));
#126012=DIRECTION('',(0.484112382334803,0.215535096873139,0.848044705947751));
#126013=DIRECTION('center_axis',(1.4081690688991E-16,6.98296267768627E-15,
-1.));
#126014=DIRECTION('ref_axis',(-1.,8.44830660832796E-31,-1.4081690688991E-16));
#126015=DIRECTION('',(-0.503986741943985,-0.163760619987452,-0.848044705947754));
#126016=DIRECTION('center_axis',(1.4081690688991E-16,6.98296267768627E-15,
-1.));
#126017=DIRECTION('ref_axis',(-1.,2.43183251313894E-12,-1.40816906872929E-16));
#126018=DIRECTION('',(0.503989916507249,0.163750849686371,0.848044705947751));
#126019=DIRECTION('center_axis',(1.4081690688991E-16,6.98296267768627E-15,
-1.));
#126020=DIRECTION('ref_axis',(-1.,8.44830660832796E-31,-1.4081690688991E-16));
#126021=DIRECTION('',(-0.518343495789664,-0.110182562533935,-0.84804470594775));
#126022=DIRECTION('center_axis',(1.4081690688991E-16,6.98296267768627E-15,
-1.));
#126023=DIRECTION('ref_axis',(-1.,2.52153853352866E-12,-1.40816906872303E-16));
#126024=DIRECTION('',(0.518345631687777,0.110172513923356,0.848044705947751));
#126025=DIRECTION('center_axis',(1.4081690688991E-16,6.98296267768627E-15,
-1.));
#126026=DIRECTION('ref_axis',(-1.,8.44830660832796E-31,-1.4081690688991E-16));
#126027=DIRECTION('',(-0.527021169825118,-0.0553973218681055,-0.84804470594775));
#126028=DIRECTION('center_axis',(1.4081690688991E-16,6.98296267768627E-15,
-1.));
#126029=DIRECTION('ref_axis',(-1.,8.43549292198398E-31,-1.4081690688991E-16));
#126030=DIRECTION('',(0.52702224365674,0.0553871050427153,0.848044705947748));
#126031=DIRECTION('center_axis',(1.4081690688991E-16,6.98296267768627E-15,
-1.));
#126032=DIRECTION('ref_axis',(-1.,8.44830660832796E-31,-1.4081690688991E-16));
#126033=DIRECTION('',(-0.5299246896377,-5.13655125503461E-6,-0.848044705947749));
#126034=DIRECTION('center_axis',(1.4081690688991E-16,6.98296267768627E-15,
-1.));
#126035=DIRECTION('ref_axis',(-1.,8.43549292198398E-31,-1.4081690688991E-16));
#126036=DIRECTION('',(-0.529919264233204,5.85699181126825E-15,-0.848048096156427));
#126037=DIRECTION('center_axis',(1.4081690688991E-16,6.98296267768627E-15,
-1.));
#126038=DIRECTION('ref_axis',(-1.,8.43549292198398E-31,-1.4081690688991E-16));
#126039=DIRECTION('',(0.5299246896377,-5.13655126669649E-6,0.848044705947748));
#126040=DIRECTION('center_axis',(1.4081690688991E-16,6.98296267768627E-15,
-1.));
#126041=DIRECTION('ref_axis',(-1.,8.44830660832796E-31,-1.4081690688991E-16));
#126042=DIRECTION('',(-0.52702224365675,0.0553871050427198,-0.848044705947742));
#126043=DIRECTION('center_axis',(1.4081690688991E-16,6.98296267768627E-15,
-1.));
#126044=DIRECTION('ref_axis',(-1.,8.43549292198398E-31,-1.4081690688991E-16));
#126045=DIRECTION('',(0.527021169825118,-0.0553973218681105,0.84804470594775));
#126046=DIRECTION('center_axis',(1.4081690688991E-16,6.98296267768627E-15,
-1.));
#126047=DIRECTION('ref_axis',(-1.,8.44830660832796E-31,-1.4081690688991E-16));
#126048=DIRECTION('',(-0.518345631687786,0.110172513923365,-0.848044705947744));
#126049=DIRECTION('center_axis',(1.4081690688991E-16,6.98296267768627E-15,
-1.));
#126050=DIRECTION('ref_axis',(-1.,8.43549292198398E-31,-1.4081690688991E-16));
#126051=DIRECTION('',(0.518343495789664,-0.110182562533938,0.84804470594775));
#126052=DIRECTION('center_axis',(1.4081690688991E-16,6.98296267768627E-15,
-1.));
#126053=DIRECTION('ref_axis',(-1.,8.44830660832796E-31,-1.4081690688991E-16));
#126054=DIRECTION('',(-0.503989916507253,0.163750849686366,-0.848044705947749));
#126055=DIRECTION('center_axis',(1.4081690688991E-16,6.98296267768627E-15,
-1.));
#126056=DIRECTION('ref_axis',(-1.,8.43549292198398E-31,-1.4081690688991E-16));
#126057=DIRECTION('',(0.50398674194398,-0.16376061998746,0.848044705947755));
#126058=DIRECTION('center_axis',(1.4081690688991E-16,6.98296267768627E-15,
-1.));
#126059=DIRECTION('ref_axis',(-1.,8.44830660832796E-31,-1.4081690688991E-16));
#126060=DIRECTION('',(-0.484112382334807,0.215535096873148,-0.848044705947747));
#126061=DIRECTION('center_axis',(1.4081690688991E-16,6.98296267768627E-15,
-1.));
#126062=DIRECTION('ref_axis',(-1.,8.43549292198398E-31,-1.4081690688991E-16));
#126063=DIRECTION('',(0.484108203887571,-0.215544481819295,0.848044705947747));
#126064=DIRECTION('center_axis',(1.4081690688991E-16,6.98296267768627E-15,
-1.));
#126065=DIRECTION('ref_axis',(-1.,8.44830660832796E-31,-1.4081690688991E-16));
#126066=DIRECTION('',(-0.458930811594466,0.264957896434968,-0.848044705947747));
#126067=DIRECTION('center_axis',(1.4081690688991E-16,6.98296267768627E-15,
-1.));
#126068=DIRECTION('ref_axis',(-1.,8.43549292198398E-31,-1.4081690688991E-16));
#126069=DIRECTION('',(0.458925675043206,-0.264966793202741,0.848044705947743));
#126070=DIRECTION('center_axis',(1.4081690688991E-16,6.98296267768627E-15,
-1.));
#126071=DIRECTION('ref_axis',(-1.,8.44830660832796E-31,-1.4081690688991E-16));
#126072=DIRECTION('',(-0.428721098844845,0.311477761837453,-0.848044705947746));
#126073=DIRECTION('center_axis',(1.4081690688991E-16,6.98296267768627E-15,
-1.));
#126074=DIRECTION('ref_axis',(-1.,8.43549292198398E-31,-1.4081690688991E-16));
#126075=DIRECTION('',(0.428715060466697,-0.311486072951958,0.848044705947749));
#126076=DIRECTION('center_axis',(1.4081690688991E-16,6.98296267768627E-15,
-1.));
#126077=DIRECTION('ref_axis',(-1.,8.44830660832796E-31,-1.4081690688991E-16));
#126078=DIRECTION('',(-0.393814228020624,0.354585011700306,-0.848044705947755));
#126079=DIRECTION('center_axis',(1.4081690688991E-16,6.98296267768627E-15,
-1.));
#126080=DIRECTION('ref_axis',(-1.,8.43549292198398E-31,-1.4081690688991E-16));
#126081=DIRECTION('',(0.393807353973302,-0.354592646103312,0.848044705947745));
#126082=DIRECTION('center_axis',(1.4081690688991E-16,6.98296267768627E-15,
-1.));
#126083=DIRECTION('ref_axis',(-1.,8.44830660832796E-31,-1.4081690688991E-16));
#126084=DIRECTION('',(-0.354592646103293,0.393807353973316,-0.848044705947747));
#126085=DIRECTION('center_axis',(1.4081690688991E-16,6.98296267768627E-15,
-1.));
#126086=DIRECTION('ref_axis',(-1.,8.43549292198398E-31,-1.4081690688991E-16));
#126087=DIRECTION('',(0.35458501170032,-0.393814228020626,0.848044705947748));
#126088=DIRECTION('center_axis',(1.4081690688991E-16,6.98296267768627E-15,
-1.));
#126089=DIRECTION('ref_axis',(-1.,8.44830660832796E-31,-1.4081690688991E-16));
#126090=DIRECTION('',(-0.311486072951978,0.428715060466679,-0.84804470594775));
#126091=DIRECTION('center_axis',(1.4081690688991E-16,6.98296267768627E-15,
-1.));
#126092=DIRECTION('ref_axis',(-1.,3.5118574714943E-12,-1.40816906865387E-16));
#126093=DIRECTION('',(0.31147776183744,-0.428721098844837,0.848044705947755));
#126094=DIRECTION('center_axis',(1.4081690688991E-16,6.98296267768627E-15,
-1.));
#126095=DIRECTION('ref_axis',(-1.,-1.95399252334028E-14,-1.40816906890047E-16));
#126096=DIRECTION('',(-0.264966793202737,0.4589256750432,-0.848044705947748));
#126097=DIRECTION('center_axis',(1.4081690688991E-16,6.98296267768627E-15,
-1.));
#126098=DIRECTION('ref_axis',(-1.,-3.60245167030371E-12,-1.40816906915066E-16));
#126099=DIRECTION('',(0.264957896434972,-0.458930811594474,0.848044705947742));
#126100=DIRECTION('center_axis',(1.4081690688991E-16,6.98296267768627E-15,
-1.));
#126101=DIRECTION('ref_axis',(-1.,1.95399252334028E-14,-1.40816906889774E-16));
#126102=DIRECTION('',(-0.215544481819303,0.48410820388756,-0.848044705947752));
#126103=DIRECTION('center_axis',(1.4081690688991E-16,6.98296267768627E-15,
-1.));
#126104=DIRECTION('ref_axis',(-1.,1.84652293455656E-12,-1.40816906877016E-16));
#126105=DIRECTION('',(0.215535096873159,-0.484112382334816,0.848044705947739));
#126106=DIRECTION('center_axis',(1.4081690688991E-16,6.98296267768627E-15,
-1.));
#126107=DIRECTION('ref_axis',(-1.,2.1316282072803E-14,-1.40816906889762E-16));
#126108=DIRECTION('',(-0.16376061998747,0.503986741944006,-0.848044705947738));
#126109=DIRECTION('center_axis',(1.4081690688991E-16,6.98296267768627E-15,
-1.));
#126110=DIRECTION('ref_axis',(-1.,1.89093185554157E-12,-1.40816906876706E-16));
#126111=DIRECTION('',(0.163750849686377,-0.503989916507272,0.848044705947736));
#126112=DIRECTION('center_axis',(1.4081690688991E-16,6.98296267768627E-15,
-1.));
#126113=DIRECTION('ref_axis',(-1.,1.06581410364015E-14,-1.40816906889836E-16));
#126114=DIRECTION('',(-0.110182562533946,0.518343495789671,-0.848044705947745));
#126115=DIRECTION('center_axis',(1.4081690688991E-16,6.98296267768627E-15,
-1.));
#126116=DIRECTION('ref_axis',(-1.,1.93622895494627E-12,-1.4081690687639E-16));
#126117=DIRECTION('',(0.110172513923365,-0.51834563168779,0.848044705947742));
#126118=DIRECTION('center_axis',(1.4081690688991E-16,6.98296267768627E-15,
-1.));
#126119=DIRECTION('ref_axis',(-1.,1.06581410364015E-14,-1.40816906889836E-16));
#126120=DIRECTION('',(-0.0553973218681178,0.527021169825125,-0.848044705947745));
#126121=DIRECTION('center_axis',(1.4081690688991E-16,6.98296267768627E-15,
-1.));
#126122=DIRECTION('ref_axis',(-1.,1.98152605435098E-12,-1.40816906876074E-16));
#126123=DIRECTION('',(0.0553871050427273,-0.527022243656745,0.848044705947745));
#126124=DIRECTION('center_axis',(1.4081690688991E-16,6.98296267768627E-15,
-1.));
#126125=DIRECTION('ref_axis',(-1.,1.15463194561016E-14,-1.4081690688983E-16));
#126126=DIRECTION('',(-5.13655126618054E-6,0.529924689637707,-0.848044705947744));
#126127=DIRECTION('',(-5.1365512553442E-6,-0.529924689637711,0.848044705947741));
#126128=DIRECTION('center_axis',(1.4081690688991E-16,6.98296267768627E-15,
-1.));
#126129=DIRECTION('ref_axis',(-1.,1.15463194561016E-14,-1.4081690688983E-16));
#126130=DIRECTION('',(0.0553871050427141,0.527022243656745,-0.848044705947745));
#126131=DIRECTION('center_axis',(1.4081690688991E-16,6.98296267768627E-15,
-1.));
#126132=DIRECTION('ref_axis',(-1.,2.07123207474069E-12,-1.40816906875447E-16));
#126133=DIRECTION('',(-0.0553973218681087,-0.52702116982513,0.848044705947743));
#126134=DIRECTION('center_axis',(1.4081690688991E-16,6.98296267768627E-15,
-1.));
#126135=DIRECTION('ref_axis',(-1.,1.15463194561016E-14,-1.4081690688983E-16));
#126136=DIRECTION('',(0.110172513923356,0.518345631687781,-0.848044705947748));
#126137=DIRECTION('center_axis',(1.4081690688991E-16,6.98296267768627E-15,
-1.));
#126138=DIRECTION('ref_axis',(-1.,2.1165291741454E-12,-1.40816906875131E-16));
#126139=DIRECTION('',(-0.110182562533934,-0.518343495789662,0.848044705947752));
#126140=DIRECTION('center_axis',(1.4081690688991E-16,6.98296267768627E-15,
-1.));
#126141=DIRECTION('ref_axis',(-1.,1.15463194561016E-14,-1.4081690688983E-16));
#126142=DIRECTION('',(0.163750849686359,0.503989916507255,-0.84804470594775));
#126143=DIRECTION('center_axis',(1.4081690688991E-16,6.98296267768627E-15,
-1.));
#126144=DIRECTION('ref_axis',(-1.,4.32276436868051E-12,-1.40816906859725E-16));
#126145=DIRECTION('',(-0.16376061998747,-0.503986741943991,0.848044705947747));
#126146=DIRECTION('center_axis',(1.4081690688991E-16,6.98296267768627E-15,
-1.));
#126147=DIRECTION('ref_axis',(-1.,1.15463194561016E-14,-1.4081690688983E-16));
#126148=DIRECTION('',(0.215535096873149,0.484112382334808,-0.848044705947746));
#126149=DIRECTION('center_axis',(1.4081690688991E-16,6.98296267768627E-15,
-1.));
#126150=DIRECTION('ref_axis',(-1.,2.20623519453511E-12,-1.40816906874504E-16));
#126151=DIRECTION('',(-0.215544481819284,-0.484108203887573,0.848044705947749));
#126152=DIRECTION('center_axis',(1.4081690688991E-16,6.98296267768627E-15,
-1.));
#126153=DIRECTION('ref_axis',(-1.,1.24344978758018E-14,-1.40816906889824E-16));
#126154=DIRECTION('',(0.264957896434972,0.458930811594474,-0.848044705947742));
#126155=DIRECTION('center_axis',(1.4081690688991E-16,6.98296267768627E-15,
-1.));
#126156=DIRECTION('ref_axis',(-1.,4.50306458787963E-12,-1.40816906858466E-16));
#126157=DIRECTION('',(-0.264966793202729,-0.458925675043209,0.848044705947745));
#126158=DIRECTION('center_axis',(1.4081690688991E-16,6.98296267768627E-15,
-1.));
#126159=DIRECTION('ref_axis',(-1.,1.86517468137026E-14,-1.4081690688978E-16));
#126160=DIRECTION('',(0.311477761837426,0.428721098844875,-0.848044705947742));
#126161=DIRECTION('center_axis',(1.4081690688991E-16,6.98296267768627E-15,
-1.));
#126162=DIRECTION('ref_axis',(-1.,1.14841469667226E-12,-1.40816906881891E-16));
#126163=DIRECTION('',(-0.311486072951947,-0.428715060466726,0.848044705947739));
#126164=DIRECTION('center_axis',(1.4081690688991E-16,6.98296267768627E-15,
-1.));
#126165=DIRECTION('ref_axis',(-1.,-1.86517468137026E-14,-1.40816906890041E-16));
#126166=DIRECTION('',(0.354585011700309,0.393814228020635,-0.848044705947748));
#126167=DIRECTION('center_axis',(1.4081690688991E-16,6.98296267768627E-15,
-1.));
#126168=DIRECTION('ref_axis',(-1.,2.34123831432953E-12,-1.40816906873562E-16));
#126169=DIRECTION('',(-0.354592646103299,-0.393807353973315,0.848044705947745));
#126170=DIRECTION('center_axis',(1.4081690688991E-16,6.98296267768627E-15,
-1.));
#126171=DIRECTION('ref_axis',(-1.,-6.21724893790088E-15,-1.40816906889954E-16));
#126172=DIRECTION('',(0.393807353973314,0.354592646103304,-0.848044705947743));
#126173=DIRECTION('center_axis',(1.4081690688991E-16,6.98296267768627E-15,
-1.));
#126174=DIRECTION('ref_axis',(-1.,1.19282361765727E-12,-1.40816906881581E-16));
#126175=DIRECTION('',(-0.393814228020621,-0.354585011700328,0.848044705947747));
#126176=DIRECTION('center_axis',(1.4081690688991E-16,6.98296267768627E-15,
-1.));
#126177=DIRECTION('ref_axis',(-1.,-1.95399252334028E-14,-1.40816906890047E-16));
#126178=DIRECTION('',(0.428715060466673,0.31148607295198,-0.848044705947753));
#126179=DIRECTION('center_axis',(1.4081690688991E-16,6.98296267768627E-15,
-1.));
#126180=DIRECTION('ref_axis',(-1.,2.43183251313894E-12,-1.40816906872929E-16));
#126181=DIRECTION('',(-0.428721098844844,-0.311477761837459,0.848044705947745));
#126182=DIRECTION('center_axis',(1.4081690688991E-16,6.98296267768627E-15,
-1.));
#126183=DIRECTION('ref_axis',(-1.,-1.33226762955019E-14,-1.40816906890003E-16));
#126184=DIRECTION('',(0.458925675043199,0.264966793202751,-0.848044705947744));
#126185=DIRECTION('center_axis',(1.4081690688991E-16,6.98296267768627E-15,
-1.));
#126186=DIRECTION('ref_axis',(-1.,4.9533710466676E-12,-1.40816906855321E-16));
#126187=DIRECTION('',(-0.458930811594451,-0.264957896434974,0.848044705947754));
#126188=DIRECTION('center_axis',(1.4081690688991E-16,6.98296267768627E-15,
-1.));
#126189=DIRECTION('ref_axis',(-1.,1.33226762955019E-14,-1.40816906889817E-16));
#126190=DIRECTION('',(0.484108203887558,0.215544481819315,-0.84804470594775));
#126191=DIRECTION('center_axis',(1.4081690688991E-16,6.98296267768627E-15,
-1.));
#126192=DIRECTION('ref_axis',(-1.,2.52153853352866E-12,-1.40816906872303E-16));
#126193=DIRECTION('',(-0.484112382334805,-0.21553509687316,0.848044705947745));
#126194=DIRECTION('center_axis',(1.4081690688991E-16,6.98296267768627E-15,
-1.));
#126195=DIRECTION('ref_axis',(-1.,4.79616346638068E-14,-1.40816906889576E-16));
#126196=DIRECTION('',(0.503986741943984,0.163760619987471,-0.848044705947751));
#126197=DIRECTION('center_axis',(1.4081690688991E-16,6.98296267768627E-15,
-1.));
#126198=DIRECTION('ref_axis',(-1.,-7.70050689880008E-12,-1.40816906943683E-16));
#126199=DIRECTION('',(-0.503989916507243,-0.163750849686383,0.848044705947753));
#126200=DIRECTION('center_axis',(1.4081690688991E-16,6.98296267768627E-15,
-1.));
#126201=DIRECTION('ref_axis',(-1.,-7.105427357601E-15,-1.4081690688996E-16));
#126202=DIRECTION('',(0.518343495789668,0.110182562533952,-0.848044705947745));
#126203=DIRECTION('center_axis',(1.4081690688991E-16,6.98296267768627E-15,
-1.));
#126204=DIRECTION('ref_axis',(-1.,2.28528307388842E-12,-1.40816906873952E-16));
#126205=DIRECTION('',(-0.518345631687771,-0.110172513923371,0.848044705947753));
#126206=DIRECTION('center_axis',(1.4081690688991E-16,6.98296267768627E-15,
-1.));
#126207=DIRECTION('ref_axis',(-1.,4.35207425653061E-14,-1.40816906889607E-16));
#126208=DIRECTION('',(0.527021169825113,0.0553973218681212,-0.848044705947752));
#126209=DIRECTION('center_axis',(1.4081690688991E-16,6.98296267768627E-15,
-1.));
#126210=DIRECTION('ref_axis',(-1.,2.65654165332307E-12,-1.4081690687136E-16));
#126211=DIRECTION('',(-0.527022243656726,-0.0553871050427333,0.848044705947756));
#126212=DIRECTION('center_axis',(1.4081690688991E-16,6.98296267768627E-15,
-1.));
#126213=DIRECTION('ref_axis',(-1.,-3.5527136788005E-15,-1.40816906889935E-16));
#126214=DIRECTION('',(0.529924689637695,5.13655126659336E-6,-0.848044705947752));
#126215=DIRECTION('center_axis',(1.4081690688991E-16,6.98296267768627E-15,
-1.));
#126216=DIRECTION('ref_axis',(1.,-8.91767816654029E-31,1.4081690688991E-16));
#126217=DIRECTION('center_axis',(-1.4081690688991E-16,-6.98296267768627E-15,
1.));
#126218=DIRECTION('ref_axis',(-1.,8.91767816654029E-31,-1.4081690688991E-16));
#126219=DIRECTION('',(-0.529919264233204,5.98678459741819E-15,-0.848048096156427));
#126220=DIRECTION('center_axis',(-1.4081690688991E-16,-6.98296267768627E-15,
1.));
#126221=DIRECTION('ref_axis',(-1.,8.91767816654029E-31,-1.4081690688991E-16));
#126222=DIRECTION('center_axis',(-1.4081690688991E-16,-6.98296267768627E-15,
1.));
#126223=DIRECTION('ref_axis',(-1.,1.21498023491345E-30,-1.4081690688991E-16));
#126224=DIRECTION('',(-1.40816906889911E-16,-6.98296267768627E-15,1.));
#126225=DIRECTION('center_axis',(-1.4081690688991E-16,-6.98296267768627E-15,
1.));
#126226=DIRECTION('ref_axis',(-1.,8.91767816654029E-31,-1.4081690688991E-16));
#126227=DIRECTION('center_axis',(-1.4081690688991E-16,-6.98296267768627E-15,
1.));
#126228=DIRECTION('ref_axis',(-1.,9.83319205199467E-31,-1.40816906889911E-16));
#126229=DIRECTION('center_axis',(-1.4081690688991E-16,-6.98296267768627E-15,
1.));
#126230=DIRECTION('ref_axis',(-1.,7.97077743482043E-31,-1.4081690688991E-16));
#126231=DIRECTION('',(-0.994521895368275,0.10452846326764,5.89872860613779E-16));
#126232=DIRECTION('center_axis',(-1.4081690688991E-16,-6.98296267768627E-15,
1.));
#126233=DIRECTION('ref_axis',(-1.,8.46073526001725E-31,-1.4081690688991E-16));
#126234=DIRECTION('',(1.,-9.83319205199467E-31,1.40816906889911E-16));
#126235=DIRECTION('center_axis',(-1.4081690688991E-16,-6.98296267768627E-15,
1.));
#126236=DIRECTION('ref_axis',(-1.,7.97077743482043E-31,-1.4081690688991E-16));
#126237=DIRECTION('center_axis',(-1.4081690688991E-16,-6.98296267768627E-15,
1.));
#126238=DIRECTION('ref_axis',(-1.,7.97077743482043E-31,-1.4081690688991E-16));
#126239=DIRECTION('center_axis',(1.4081690688991E-16,6.98296267768627E-15,
-1.));
#126240=DIRECTION('ref_axis',(1.,-7.97077743482043E-31,1.4081690688991E-16));
#126241=DIRECTION('center_axis',(1.4081690688991E-16,6.98296267768627E-15,
-1.));
#126242=DIRECTION('ref_axis',(-1.,7.97577417048809E-31,-1.40816906889911E-16));
#126243=DIRECTION('',(-0.497265611060805,0.0522695260941841,0.866022406579768));
#126244=DIRECTION('',(0.500005191251968,4.7780011719149E-6,-0.866022406579792));
#126245=DIRECTION('center_axis',(-1.4081690688991E-16,-6.98296267768627E-15,
1.));
#126246=DIRECTION('ref_axis',(-1.,9.83319205199467E-31,-1.40816906889911E-16));
#126247=DIRECTION('center_axis',(1.4081690688991E-16,6.98296267768627E-15,
-1.));
#126248=DIRECTION('ref_axis',(-1.,7.98707387273907E-31,-1.4081690688991E-16));
#126249=DIRECTION('',(-0.994521895368275,0.10452846326764,5.89872860613779E-16));
#126250=DIRECTION('center_axis',(-1.4081690688991E-16,-6.98296267768627E-15,
1.));
#126251=DIRECTION('ref_axis',(-1.,7.98248735348668E-31,-1.4081690688991E-16));
#126252=DIRECTION('',(1.,-9.83319205199467E-31,1.40816906889911E-16));
#126253=DIRECTION('center_axis',(-1.4081690688991E-16,-6.98296267768627E-15,
1.));
#126254=DIRECTION('ref_axis',(-1.,7.99150043815584E-31,-1.4081690688991E-16));
#126255=DIRECTION('center_axis',(-1.4081690688991E-16,-6.98296267768627E-15,
1.));
#126256=DIRECTION('ref_axis',(-1.,7.99858039355471E-31,-1.4081690688991E-16));
#126257=DIRECTION('',(-0.497266395846506,0.0522601510654359,-0.86602252174666));
#126258=DIRECTION('center_axis',(-1.4081690688991E-16,-6.98296267768627E-15,
1.));
#126259=DIRECTION('ref_axis',(1.,-3.37507799486047E-14,1.40816906889675E-16));
#126260=DIRECTION('',(0.500004991781248,-4.62770265895208E-6,0.866022521746645));
#126261=DIRECTION('center_axis',(-1.4081690688991E-16,-6.98296267768627E-15,
1.));
#126262=DIRECTION('ref_axis',(-1.,7.99858039355471E-31,-1.4081690688991E-16));
#126263=DIRECTION('center_axis',(-1.4081690688991E-16,-6.98296267768627E-15,
1.));
#126264=DIRECTION('ref_axis',(-1.,7.99858039355471E-31,-1.4081690688991E-16));
#126265=DIRECTION('center_axis',(-1.4081690688991E-16,-6.98296267768627E-15,
1.));
#126266=DIRECTION('ref_axis',(-1.,9.83319205199467E-31,-1.40816906889911E-16));
#126267=DIRECTION('center_axis',(1.4081690688991E-16,6.98296267768627E-15,
-1.));
#126268=DIRECTION('ref_axis',(-1.,8.01265634860448E-31,-1.4081690688991E-16));
#126269=DIRECTION('',(-0.994521895368275,0.10452846326764,5.89872860613779E-16));
#126270=DIRECTION('',(1.,-9.83319205199467E-31,1.40816906889911E-16));
#126271=DIRECTION('center_axis',(-1.4081690688991E-16,-6.98296267768627E-15,
1.));
#126272=DIRECTION('ref_axis',(-1.,8.32577322149061E-31,-1.39145123902276E-16));
#126273=DIRECTION('center_axis',(-0.103464010407632,-0.994633197962203,
-7.86457232282242E-6));
#126274=DIRECTION('ref_axis',(-0.843493966781849,0.0877379732620279,0.529924500330464));
#126275=DIRECTION('center_axis',(0.0010702559647624,0.999999427244995,-7.86457193703672E-6));
#126276=DIRECTION('ref_axis',(1.47312952164193E-6,7.86299981466101E-6,0.999999999968002));
#126277=DIRECTION('center_axis',(-1.4081690688991E-16,-6.98296267768627E-15,
1.));
#126278=DIRECTION('ref_axis',(-1.,8.07722881720021E-31,-1.42096112075504E-16));
#126279=DIRECTION('center_axis',(-0.103509373496232,-0.994628478127866,
9.77051633950369E-6));
#126280=DIRECTION('ref_axis',(0.869950553189692,-0.0905391058403728,-0.484756336027261));
#126281=DIRECTION('center_axis',(0.00102464806169094,0.999999475000305,
9.77058601219822E-6));
#126282=DIRECTION('ref_axis',(0.874641264346837,-0.000891463458120753,-0.484769908301526));
#126283=DIRECTION('center_axis',(-1.4081690688991E-16,-6.98296267768627E-15,
1.));
#126284=DIRECTION('ref_axis',(-1.,8.24049048117772E-31,-1.37719829560012E-16));
#126285=DIRECTION('center_axis',(0.107112171226385,0.994246942387259,-1.81316452017406E-5));
#126286=DIRECTION('ref_axis',(0.861994650485032,-0.092855284670664,0.498340364253106));
#126287=DIRECTION('center_axis',(0.00259831235053356,-0.999996624215829,
-1.81624798012333E-5));
#126288=DIRECTION('ref_axis',(0.865241946199119,0.00223907064273735,0.501349539842431));
#126289=DIRECTION('center_axis',(-1.4081690688991E-16,-6.98296267768627E-15,
1.));
#126290=DIRECTION('ref_axis',(-1.,8.26087817385229E-31,-1.38060560438432E-16));
#126291=DIRECTION('center_axis',(0.10712560498354,0.994245495043206,-1.85257092162474E-5));
#126292=DIRECTION('ref_axis',(0.860265387811452,-0.092699175819097,-0.501348506865306));
#126293=DIRECTION('center_axis',(0.00261182427502986,-0.999996589010146,
-1.84940601812351E-5));
#126294=DIRECTION('ref_axis',(0.866979057021848,0.00227362102099719,-0.498339387699748));
#126295=DIRECTION('center_axis',(-1.4081690688991E-16,-6.98296267768627E-15,
1.));
#126296=DIRECTION('ref_axis',(-1.,9.83319205199467E-31,-1.40816906889911E-16));
#126297=DIRECTION('center_axis',(-1.4081690688991E-16,-6.98296267768627E-15,
1.));
#126298=DIRECTION('ref_axis',(-1.,8.46073526001725E-31,-1.4081690688991E-16));
#126299=DIRECTION('',(0.994521895368275,-0.10452846326764,-5.89872860613779E-16));
#126300=DIRECTION('center_axis',(-1.4081690688991E-16,-6.98296267768627E-15,
1.));
#126301=DIRECTION('ref_axis',(-1.,7.97077743482043E-31,-1.4081690688991E-16));
#126302=DIRECTION('center_axis',(-1.4081690688991E-16,-6.98296267768627E-15,
1.));
#126303=DIRECTION('ref_axis',(-1.,7.97077743482043E-31,-1.4081690688991E-16));
#126304=DIRECTION('center_axis',(-1.4081690688991E-16,-6.98296267768627E-15,
1.));
#126305=DIRECTION('ref_axis',(-1.,7.97077743482043E-31,-1.4081690688991E-16));
#126306=DIRECTION('',(-0.978147600733808,0.207911690817747,1.31409985761785E-15));
#126307=DIRECTION('center_axis',(1.4081690688991E-16,6.98296267768627E-15,
-1.));
#126308=DIRECTION('ref_axis',(1.,-7.97077743482043E-31,1.4081690688991E-16));
#126309=DIRECTION('',(0.497266609935019,-0.0522600224406333,-0.866022406579783));
#126310=DIRECTION('center_axis',(1.4081690688991E-16,6.98296267768627E-15,
-1.));
#126311=DIRECTION('ref_axis',(-1.,7.97577417048809E-31,-1.40816906889911E-16));
#126312=DIRECTION('',(-0.489077884775291,0.103961598321232,0.866022406579773));
#126313=DIRECTION('center_axis',(-1.4081690688991E-16,-6.98296267768627E-15,
1.));
#126314=DIRECTION('ref_axis',(-1.,9.83319205199467E-31,-1.40816906889911E-16));
#126315=DIRECTION('center_axis',(-1.4081690688991E-16,-6.98296267768627E-15,
1.));
#126316=DIRECTION('ref_axis',(-1.,7.98248735348668E-31,-1.4081690688991E-16));
#126317=DIRECTION('',(0.994521895368275,-0.10452846326764,-5.89872860613779E-16));
#126318=DIRECTION('center_axis',(1.4081690688991E-16,6.98296267768627E-15,
-1.));
#126319=DIRECTION('ref_axis',(-1.,7.98707387273907E-31,-1.4081690688991E-16));
#126320=DIRECTION('',(-0.978147600733808,0.207911690817747,1.31409985761785E-15));
#126321=DIRECTION('center_axis',(-1.4081690688991E-16,-6.98296267768627E-15,
1.));
#126322=DIRECTION('ref_axis',(-1.,7.99150043815584E-31,-1.4081690688991E-16));
#126323=DIRECTION('center_axis',(-1.4081690688991E-16,-6.98296267768627E-15,
1.));
#126324=DIRECTION('ref_axis',(1.,-1.95399252334028E-14,1.40816906889774E-16));
#126325=DIRECTION('',(0.497265428393217,-0.0522693557686642,0.866022521746657));
#126326=DIRECTION('center_axis',(-1.4081690688991E-16,-6.98296267768627E-15,
1.));
#126327=DIRECTION('ref_axis',(-1.,7.99858039355471E-31,-1.4081690688991E-16));
#126328=DIRECTION('center_axis',(-1.4081690688991E-16,-6.98296267768627E-15,
1.));
#126329=DIRECTION('ref_axis',(-1.,7.99858039355471E-31,-1.4081690688991E-16));
#126330=DIRECTION('center_axis',(-1.4081690688991E-16,-6.98296267768627E-15,
1.));
#126331=DIRECTION('ref_axis',(-1.,7.99858039355471E-31,-1.4081690688991E-16));
#126332=DIRECTION('',(-0.489079645219224,0.103952356682307,-0.866022521746653));
#126333=DIRECTION('center_axis',(-1.4081690688991E-16,-6.98296267768627E-15,
1.));
#126334=DIRECTION('ref_axis',(-1.,9.83319205199467E-31,-1.40816906889911E-16));
#126335=DIRECTION('',(0.994521895368275,-0.10452846326764,-5.89872860613779E-16));
#126336=DIRECTION('center_axis',(1.4081690688991E-16,6.98296267768627E-15,
-1.));
#126337=DIRECTION('ref_axis',(-1.,8.01265634860448E-31,-1.4081690688991E-16));
#126338=DIRECTION('',(-0.978147600733808,0.207911690817747,1.31409985761785E-15));
#126339=DIRECTION('center_axis',(-1.4081690688991E-16,-6.98296267768627E-15,
1.));
#126340=DIRECTION('ref_axis',(-1.,8.32577322149061E-31,-1.39145123902276E-16));
#126341=DIRECTION('center_axis',(0.105592796389084,0.994409453539578,-7.86457209645399E-6));
#126342=DIRECTION('ref_axis',(2.28696687445887E-6,7.66594167224769E-6,0.999999999968002));
#126343=DIRECTION('center_axis',(-0.206864703430973,-0.97836955922216,-7.8645723370883E-6));
#126344=DIRECTION('ref_axis',(-0.829702103060295,0.175426463587553,0.52992450033046));
#126345=DIRECTION('center_axis',(-1.4081690688991E-16,-6.98296267768627E-15,
1.));
#126346=DIRECTION('ref_axis',(-1.,8.07722881720021E-31,-1.42096112075504E-16));
#126347=DIRECTION('center_axis',(0.105547443322659,0.994414268357301,9.77058606584058E-6));
#126348=DIRECTION('ref_axis',(0.869756704679887,-0.0923114872006333,-0.484769908302064));
#126349=DIRECTION('center_axis',(-0.206909324657823,-0.978360123509835,
9.77051813555105E-6));
#126350=DIRECTION('ref_axis',(0.855720959435949,-0.18097771758911,-0.484756336026932));
#126351=DIRECTION('center_axis',(-1.4081690688991E-16,-6.98296267768627E-15,
1.));
#126352=DIRECTION('ref_axis',(-1.,8.24049048117772E-31,-1.37719829560012E-16));
#126353=DIRECTION('center_axis',(-0.101944031878512,-0.994790135674091,
-1.81624797208528E-5));
#126354=DIRECTION('ref_axis',(0.860736106901394,-0.0882156062115827,0.501349539839177));
#126355=DIRECTION('center_axis',(0.210452504541382,0.977604082951531,-1.81316451947357E-5));
#126356=DIRECTION('ref_axis',(0.847566533384697,-0.182449589865756,0.498340364253253));
#126357=DIRECTION('center_axis',(-1.4081690688991E-16,-6.98296267768627E-15,
1.));
#126358=DIRECTION('ref_axis',(-1.,8.26087817385229E-31,-1.38060560438432E-16));
#126359=DIRECTION('center_axis',(-0.101930590292343,-0.994791513042117,
-1.84940577700706E-5));
#126360=DIRECTION('ref_axis',(0.862467313147314,-0.0883628226287556,-0.49833938769631));
#126361=DIRECTION('center_axis',(0.210465713413695,0.977601239327192,-1.85257175165895E-5));
#126362=DIRECTION('ref_axis',(0.845863061615653,-0.182113579025916,-0.501348506857821));
#126363=DIRECTION('center_axis',(-1.4081690688991E-16,-6.98296267768627E-15,
1.));
#126364=DIRECTION('ref_axis',(-1.,9.83319205199467E-31,-1.40816906889911E-16));
#126365=DIRECTION('center_axis',(-1.4081690688991E-16,-6.98296267768627E-15,
1.));
#126366=DIRECTION('ref_axis',(-1.,8.46073526001725E-31,-1.4081690688991E-16));
#126367=DIRECTION('',(0.978147600733808,-0.207911690817747,-1.31409985761785E-15));
#126368=DIRECTION('center_axis',(-1.4081690688991E-16,-6.98296267768627E-15,
1.));
#126369=DIRECTION('ref_axis',(-1.,7.97077743482043E-31,-1.4081690688991E-16));
#126370=DIRECTION('center_axis',(-1.4081690688991E-16,-6.98296267768627E-15,
1.));
#126371=DIRECTION('ref_axis',(-1.,7.97077743482043E-31,-1.4081690688991E-16));
#126372=DIRECTION('center_axis',(-1.4081690688991E-16,-6.98296267768627E-15,
1.));
#126373=DIRECTION('ref_axis',(-1.,7.97077743482043E-31,-1.4081690688991E-16));
#126374=DIRECTION('',(-0.951056516295158,0.309016994374935,2.02392930158878E-15));
#126375=DIRECTION('center_axis',(1.4081690688991E-16,6.98296267768627E-15,
-1.));
#126376=DIRECTION('ref_axis',(1.,-7.97077743482043E-31,1.4081690688991E-16));
#126377=DIRECTION('',(0.489079871579877,-0.103952251140467,-0.866022406579784));
#126378=DIRECTION('center_axis',(1.4081690688991E-16,6.98296267768627E-15,
-1.));
#126379=DIRECTION('ref_axis',(-1.,7.97577417048809E-31,-1.40816906889911E-16));
#126380=DIRECTION('',(-0.475531718838029,0.154514645521697,0.866022406579792));
#126381=DIRECTION('center_axis',(-1.4081690688991E-16,-6.98296267768627E-15,
1.));
#126382=DIRECTION('ref_axis',(-1.,9.83319205199467E-31,-1.40816906889911E-16));
#126383=DIRECTION('center_axis',(-1.4081690688991E-16,-6.98296267768627E-15,
1.));
#126384=DIRECTION('ref_axis',(-1.,7.98248735348668E-31,-1.4081690688991E-16));
#126385=DIRECTION('',(0.978147600733808,-0.207911690817747,-1.31409985761785E-15));
#126386=DIRECTION('center_axis',(1.4081690688991E-16,6.98296267768627E-15,
-1.));
#126387=DIRECTION('ref_axis',(-1.,7.98707387273907E-31,-1.4081690688991E-16));
#126388=DIRECTION('',(-0.951056516295158,0.309016994374935,2.02392930158878E-15));
#126389=DIRECTION('center_axis',(-1.4081690688991E-16,-6.98296267768627E-15,
1.));
#126390=DIRECTION('ref_axis',(-1.,7.99150043815584E-31,-1.4081690688991E-16));
#126391=DIRECTION('center_axis',(-1.4081690688991E-16,-6.98296267768627E-15,
1.));
#126392=DIRECTION('ref_axis',(1.,-1.4210854715202E-14,1.40816906889811E-16));
#126393=DIRECTION('',(0.489077720912262,-0.103961409834802,0.866022521746651));
#126394=DIRECTION('center_axis',(-1.4081690688991E-16,-6.98296267768627E-15,
1.));
#126395=DIRECTION('ref_axis',(-1.,7.99858039355471E-31,-1.4081690688991E-16));
#126396=DIRECTION('center_axis',(-1.4081690688991E-16,-6.98296267768627E-15,
1.));
#126397=DIRECTION('ref_axis',(-1.,7.99858039355471E-31,-1.4081690688991E-16));
#126398=DIRECTION('center_axis',(-1.4081690688991E-16,-6.98296267768627E-15,
1.));
#126399=DIRECTION('ref_axis',(-1.,7.99858039355471E-31,-1.4081690688991E-16));
#126400=DIRECTION('',(-0.475534435652402,0.154505638525938,-0.86602252174666));
#126401=DIRECTION('center_axis',(-1.4081690688991E-16,-6.98296267768627E-15,
1.));
#126402=DIRECTION('ref_axis',(-1.,9.83319205199467E-31,-1.40816906889911E-16));
#126403=DIRECTION('',(0.978147600733808,-0.207911690817747,-1.31409985761785E-15));
#126404=DIRECTION('center_axis',(1.4081690688991E-16,6.98296267768627E-15,
-1.));
#126405=DIRECTION('ref_axis',(-1.,8.01265634860448E-31,-1.4081690688991E-16));
#126406=DIRECTION('',(-0.951056516295158,0.309016994374935,2.02392930158878E-15));
#126407=DIRECTION('center_axis',(-1.4081690688991E-16,-6.98296267768627E-15,
1.));
#126408=DIRECTION('ref_axis',(-1.,8.32577322149061E-31,-1.39145123902276E-16));
#126409=DIRECTION('center_axis',(0.20895844003943,0.977924521767624,-7.86457210795472E-6));
#126410=DIRECTION('ref_axis',(3.07574773432243E-6,7.38489372014646E-6,0.999999999968002));
#126411=DIRECTION('center_axis',(-0.307998943474314,-0.951386698854286,
-7.86457232392837E-6));
#126412=DIRECTION('ref_axis',(-0.806819849471267,0.261192944867688,0.529924500330479));
#126413=DIRECTION('center_axis',(-1.4081690688991E-16,-6.98296267768627E-15,
1.));
#126414=DIRECTION('ref_axis',(-1.,8.07722881720021E-31,-1.42096112075504E-16));
#126415=DIRECTION('center_axis',(0.208913838706166,0.977934050895862,9.77058399236075E-6));
#126416=DIRECTION('ref_axis',(0.855342908547872,-0.182720126971788,-0.484769908303187));
#126417=DIRECTION('center_axis',(-0.308042333963518,-0.951372650642663,
9.77051317041121E-6));
#126418=DIRECTION('ref_axis',(0.832115907779501,-0.269433499591963,-0.484756336026591));
#126419=DIRECTION('center_axis',(-1.4081690688991E-16,-6.98296267768627E-15,
1.));
#126420=DIRECTION('ref_axis',(-1.,8.24049048117772E-31,-1.37719829560012E-16));
#126421=DIRECTION('center_axis',(-0.205369455961149,-0.978684518232687,
-1.81624796820396E-5));
#126422=DIRECTION('ref_axis',(0.846799862691371,-0.177703774423439,0.50134953984375));
#126423=DIRECTION('center_axis',(0.311487076176625,0.950250388606172,-1.81316452791439E-5));
#126424=DIRECTION('ref_axis',(0.823852299981103,-0.270044939174595,0.498340364251217));
#126425=DIRECTION('center_axis',(-1.4081690688991E-16,-6.98296267768627E-15,
1.));
#126426=DIRECTION('ref_axis',(-1.,8.26087817385229E-31,-1.38060560438432E-16));
#126427=DIRECTION('center_axis',(-0.205356231986263,-0.978687293083125,
-1.84940625565383E-5));
#126428=DIRECTION('ref_axis',(0.848506196903525,-0.17803114470241,-0.498339387699052));
#126429=DIRECTION('center_axis',(0.311499915448438,0.950246179856785,-1.85257197232984E-5));
#126430=DIRECTION('ref_axis',(0.822193282701967,-0.269532707749963,-0.501348506861979));
#126431=DIRECTION('center_axis',(-1.4081690688991E-16,-6.98296267768627E-15,
1.));
#126432=DIRECTION('ref_axis',(-1.,9.83319205199467E-31,-1.40816906889911E-16));
#126433=DIRECTION('center_axis',(-1.4081690688991E-16,-6.98296267768627E-15,
1.));
#126434=DIRECTION('ref_axis',(-1.,8.46073526001725E-31,-1.4081690688991E-16));
#126435=DIRECTION('',(0.951056516295158,-0.309016994374935,-2.02392930158878E-15));
#126436=DIRECTION('center_axis',(-1.4081690688991E-16,-6.98296267768627E-15,
1.));
#126437=DIRECTION('ref_axis',(-1.,7.97077743482043E-31,-1.4081690688991E-16));
#126438=DIRECTION('center_axis',(-1.4081690688991E-16,-6.98296267768627E-15,
1.));
#126439=DIRECTION('ref_axis',(-1.,7.97077743482043E-31,-1.4081690688991E-16));
#126440=DIRECTION('center_axis',(-1.4081690688991E-16,-6.98296267768627E-15,
1.));
#126441=DIRECTION('ref_axis',(-1.,7.97077743482043E-31,-1.4081690688991E-16));
#126442=DIRECTION('',(-0.913545457642606,0.406736643075789,2.71158415259707E-15));
#126443=DIRECTION('center_axis',(1.4081690688991E-16,6.98296267768627E-15,
-1.));
#126444=DIRECTION('ref_axis',(1.,-7.97077743482043E-31,1.4081690688991E-16));
#126445=DIRECTION('',(0.475534671805145,-0.154505557223404,-0.866022406579794));
#126446=DIRECTION('center_axis',(1.4081690688991E-16,6.98296267768627E-15,
-1.));
#126447=DIRECTION('ref_axis',(-1.,7.97577417048809E-31,-1.40816906889911E-16));
#126448=DIRECTION('',(-0.456775527877826,0.203374797931553,0.86602240657978));
#126449=DIRECTION('center_axis',(-1.4081690688991E-16,-6.98296267768627E-15,
1.));
#126450=DIRECTION('ref_axis',(-1.,9.83319205199467E-31,-1.40816906889911E-16));
#126451=DIRECTION('center_axis',(-1.4081690688991E-16,-6.98296267768627E-15,
1.));
#126452=DIRECTION('ref_axis',(-1.,7.98248735348668E-31,-1.4081690688991E-16));
#126453=DIRECTION('',(0.951056516295158,-0.309016994374935,-2.02392930158878E-15));
#126454=DIRECTION('center_axis',(1.4081690688991E-16,6.98296267768627E-15,
-1.));
#126455=DIRECTION('ref_axis',(-1.,7.98707387273907E-31,-1.4081690688991E-16));
#126456=DIRECTION('',(-0.913545457642606,0.406736643075789,2.71158415259707E-15));
#126457=DIRECTION('center_axis',(-1.4081690688991E-16,-6.98296267768627E-15,
1.));
#126458=DIRECTION('ref_axis',(-1.,7.99150043815584E-31,-1.4081690688991E-16));
#126459=DIRECTION('center_axis',(-1.4081690688991E-16,-6.98296267768627E-15,
1.));
#126460=DIRECTION('ref_axis',(1.,-2.04281036531029E-14,1.40816906889768E-16));
#126461=DIRECTION('',(0.47553157557488,-0.154514440939486,0.866022521746652));
#126462=DIRECTION('center_axis',(-1.4081690688991E-16,-6.98296267768627E-15,
1.));
#126463=DIRECTION('ref_axis',(-1.,7.99858039355471E-31,-1.4081690688991E-16));
#126464=DIRECTION('center_axis',(-1.4081690688991E-16,-6.98296267768627E-15,
1.));
#126465=DIRECTION('ref_axis',(-1.,7.99858039355471E-31,-1.4081690688991E-16));
#126466=DIRECTION('center_axis',(-1.4081690688991E-16,-6.98296267768627E-15,
1.));
#126467=DIRECTION('ref_axis',(-1.,7.99858039355471E-31,-1.4081690688991E-16));
#126468=DIRECTION('',(-0.456779171296626,0.203366124261497,-0.866022521746649));
#126469=DIRECTION('center_axis',(-1.4081690688991E-16,-6.98296267768627E-15,
1.));
#126470=DIRECTION('ref_axis',(-1.,9.83319205199467E-31,-1.40816906889911E-16));
#126471=DIRECTION('',(0.951056516295158,-0.309016994374935,-2.02392930158878E-15));
#126472=DIRECTION('center_axis',(1.4081690688991E-16,6.98296267768627E-15,
-1.));
#126473=DIRECTION('ref_axis',(-1.,8.01265634860448E-31,-1.4081690688991E-16));
#126474=DIRECTION('',(-0.913545457642606,0.406736643075789,2.71158415259707E-15));
#126475=DIRECTION('center_axis',(-1.4081690688991E-16,-6.98296267768627E-15,
1.));
#126476=DIRECTION('ref_axis',(-1.,8.32577322149061E-31,-1.39145123902276E-16));
#126477=DIRECTION('center_axis',(0.310034691293364,0.950725244291313,-7.86457215694468E-6));
#126478=DIRECTION('ref_axis',(3.83083003964029E-6,7.02293537238877E-6,0.999999999968002));
#126479=DIRECTION('center_axis',(-0.40575868264004,-0.913980246723291,-7.86457230346941E-6));
#126480=DIRECTION('ref_axis',(-0.775097908773545,0.344097741585733,0.529924500330449));
#126481=DIRECTION('center_axis',(-1.4081690688991E-16,-6.98296267768627E-15,
1.));
#126482=DIRECTION('ref_axis',(-1.,8.07722881720021E-31,-1.42096112075504E-16));
#126483=DIRECTION('center_axis',(0.309991330354408,0.950739383327335,9.77058099945129E-6));
#126484=DIRECTION('ref_axis',(0.831557796517697,-0.271126846795087,-0.484769908304534));
#126485=DIRECTION('center_axis',(-0.405800366994072,-0.913961739927889,
9.77051230122167E-6));
#126486=DIRECTION('ref_axis',(0.799394020106066,-0.354937311790806,-0.484756336026027));
#126487=DIRECTION('center_axis',(-1.4081690688991E-16,-6.98296267768627E-15,
1.));
#126488=DIRECTION('ref_axis',(-1.,8.24049048117772E-31,-1.37719829560012E-16));
#126489=DIRECTION('center_axis',(-0.306544809307814,-0.951856228406665,
-1.81624799272238E-5));
#126490=DIRECTION('ref_axis',(0.823585901983193,-0.265244982895809,0.501349539845338));
#126491=DIRECTION('center_axis',(0.409108930222443,0.912485552150549,-1.81316453655189E-5));
#126492=DIRECTION('ref_axis',(0.79111176837416,-0.354681619618438,0.498340364253942));
#126493=DIRECTION('center_axis',(-1.4081690688991E-16,-6.98296267768627E-15,
1.));
#126494=DIRECTION('ref_axis',(-1.,8.26087817385229E-31,-1.38060560438432E-16));
#126495=DIRECTION('center_axis',(-0.306531947828723,-0.951860370337109,
-1.84940671421675E-5));
#126496=DIRECTION('ref_axis',(0.825248669206747,-0.265748920299438,-0.498339387698962));
#126497=DIRECTION('center_axis',(0.409121259222292,0.912480024389117,-1.85257252778069E-5));
#126498=DIRECTION('ref_axis',(0.789515382127622,-0.353998779723841,-0.501348506867137));
#126499=DIRECTION('center_axis',(-1.4081690688991E-16,-6.98296267768627E-15,
1.));
#126500=DIRECTION('ref_axis',(-1.,9.83319205199467E-31,-1.40816906889911E-16));
#126501=DIRECTION('center_axis',(-1.4081690688991E-16,-6.98296267768627E-15,
1.));
#126502=DIRECTION('ref_axis',(-1.,8.46073526001725E-31,-1.4081690688991E-16));
#126503=DIRECTION('',(0.913545457642606,-0.406736643075789,-2.71158415259707E-15));
#126504=DIRECTION('center_axis',(-1.4081690688991E-16,-6.98296267768627E-15,
1.));
#126505=DIRECTION('ref_axis',(-1.,7.97077743482043E-31,-1.4081690688991E-16));
#126506=DIRECTION('center_axis',(-1.4081690688991E-16,-6.98296267768627E-15,
1.));
#126507=DIRECTION('ref_axis',(-1.,7.97077743482043E-31,-1.4081690688991E-16));
#126508=DIRECTION('center_axis',(-1.4081690688991E-16,-6.98296267768627E-15,
1.));
#126509=DIRECTION('ref_axis',(-1.,7.97077743482043E-31,-1.4081690688991E-16));
#126510=DIRECTION('',(-0.866025403784445,0.499999999999989,3.36953032019404E-15));
#126511=DIRECTION('center_axis',(1.4081690688991E-16,6.98296267768627E-15,
-1.));
#126512=DIRECTION('ref_axis',(1.,-7.97077743482043E-31,1.4081690688991E-16));
#126513=DIRECTION('',(0.456779414654135,-0.203366068089035,-0.866022406579779));
#126514=DIRECTION('center_axis',(1.4081690688991E-16,6.98296267768627E-15,
-1.));
#126515=DIRECTION('ref_axis',(-1.,7.97577417048809E-31,-1.40816906889911E-16));
#126516=DIRECTION('',(-0.433014808647732,0.250006733496379,0.866022406579783));
#126517=DIRECTION('center_axis',(-1.4081690688991E-16,-6.98296267768627E-15,
1.));
#126518=DIRECTION('ref_axis',(-1.,9.83319205199467E-31,-1.40816906889911E-16));
#126519=DIRECTION('center_axis',(-1.4081690688991E-16,-6.98296267768627E-15,
1.));
#126520=DIRECTION('ref_axis',(-1.,7.98248735348668E-31,-1.4081690688991E-16));
#126521=DIRECTION('',(0.913545457642606,-0.406736643075789,-2.71158415259707E-15));
#126522=DIRECTION('center_axis',(1.4081690688991E-16,6.98296267768627E-15,
-1.));
#126523=DIRECTION('ref_axis',(-1.,7.98707387273907E-31,-1.4081690688991E-16));
#126524=DIRECTION('',(-0.866025403784445,0.499999999999989,3.36953032019404E-15));
#126525=DIRECTION('center_axis',(-1.4081690688991E-16,-6.98296267768627E-15,
1.));
#126526=DIRECTION('ref_axis',(-1.,7.99150043815584E-31,-1.4081690688991E-16));
#126527=DIRECTION('center_axis',(-1.4081690688991E-16,-6.98296267768627E-15,
1.));
#126528=DIRECTION('ref_axis',(1.,-2.48689957516035E-14,1.40816906889737E-16));
#126529=DIRECTION('',(0.456775406784114,-0.203374579494981,0.866022521746661));
#126530=DIRECTION('center_axis',(-1.4081690688991E-16,-6.98296267768627E-15,
1.));
#126531=DIRECTION('ref_axis',(-1.,7.99858039355471E-31,-1.4081690688991E-16));
#126532=DIRECTION('center_axis',(-1.4081690688991E-16,-6.98296267768627E-15,
1.));
#126533=DIRECTION('ref_axis',(-1.,7.99858039355471E-31,-1.4081690688991E-16));
#126534=DIRECTION('center_axis',(-1.4081690688991E-16,-6.98296267768627E-15,
1.));
#126535=DIRECTION('ref_axis',(-1.,7.99858039355471E-31,-1.4081690688991E-16));
#126536=DIRECTION('',(-0.433019338752907,0.249998488182543,-0.866022521746657));
#126537=DIRECTION('center_axis',(-1.4081690688991E-16,-6.98296267768627E-15,
1.));
#126538=DIRECTION('ref_axis',(-1.,9.83319205199467E-31,-1.40816906889911E-16));
#126539=DIRECTION('',(0.913545457642606,-0.406736643075789,-2.71158415259707E-15));
#126540=DIRECTION('center_axis',(1.4081690688991E-16,6.98296267768627E-15,
-1.));
#126541=DIRECTION('ref_axis',(-1.,8.01265634860448E-31,-1.4081690688991E-16));
#126542=DIRECTION('',(-0.866025403784445,0.499999999999989,3.36953032019404E-15));
#126543=DIRECTION('center_axis',(-1.4081690688991E-16,-6.98296267768627E-15,
1.));
#126544=DIRECTION('ref_axis',(-1.,8.32577322149061E-31,-1.39145123902276E-16));
#126545=DIRECTION('center_axis',(0.407714137590522,0.913109622086508,-7.86457213947159E-6));
#126546=DIRECTION('ref_axis',(4.54394101111081E-6,6.58403219129901E-6,0.999999999968002));
#126547=DIRECTION('center_axis',(-0.499072844768375,-0.866560035746485,
-7.86457220438562E-6));
#126548=DIRECTION('ref_axis',(-0.734883833187544,0.423232531439973,0.529924500330466));
#126549=DIRECTION('center_axis',(-1.4081690688991E-16,-6.98296267768627E-15,
1.));
#126550=DIRECTION('ref_axis',(-1.,8.07722881720021E-31,-1.42096112075504E-16));
#126551=DIRECTION('center_axis',(0.4076724921206,0.913128216119026,9.77058401138E-6));
#126552=DIRECTION('ref_axis',(0.79866196325535,-0.356563044148319,-0.484769908303717));
#126553=DIRECTION('center_axis',(-0.499112366283222,-0.866537273132379,
9.77051426432124E-6));
#126554=DIRECTION('ref_axis',(0.757913804264544,-0.436552356526389,-0.484756336025125));
#126555=DIRECTION('center_axis',(-1.4081690688991E-16,-6.98296267768627E-15,
1.));
#126556=DIRECTION('ref_axis',(-1.,8.24049048117772E-31,-1.37719829560012E-16));
#126557=DIRECTION('center_axis',(-0.404361593575263,-0.914599202553445,
-1.81624797807593E-5));
#126558=DIRECTION('ref_axis',(0.791348561789699,-0.349880111830686,0.50134953984094));
#126559=DIRECTION('center_axis',(0.502248501217129,0.864723333035712,-1.81316454324455E-5));
#126560=DIRECTION('ref_axis',(0.749703650686919,-0.435432334018187,0.498340364247348));
#126561=DIRECTION('center_axis',(-1.4081690688991E-16,-6.98296267768627E-15,
1.));
#126562=DIRECTION('ref_axis',(-1.,8.26087817385229E-31,-1.38060560438432E-16));
#126563=DIRECTION('center_axis',(-0.404349235492276,-0.914604666189049,
-1.84940481536951E-5));
#126564=DIRECTION('ref_axis',(0.792949544396744,-0.350555095114578,-0.498339387696984));
#126565=DIRECTION('center_axis',(0.502260184874678,0.864716546821242,-1.85257139420342E-5));
#126566=DIRECTION('ref_axis',(0.74818738581782,-0.434586366991852,-0.501348506857176));
#126567=DIRECTION('center_axis',(-1.4081690688991E-16,-6.98296267768627E-15,
1.));
#126568=DIRECTION('ref_axis',(-1.,9.83319205199467E-31,-1.40816906889911E-16));
#126569=DIRECTION('center_axis',(-1.4081690688991E-16,-6.98296267768627E-15,
1.));
#126570=DIRECTION('ref_axis',(-1.,8.46073526001725E-31,-1.4081690688991E-16));
#126571=DIRECTION('',(0.866025403784445,-0.499999999999989,-3.36953032019404E-15));
#126572=DIRECTION('center_axis',(-1.4081690688991E-16,-6.98296267768627E-15,
1.));
#126573=DIRECTION('ref_axis',(-1.,7.97077743482043E-31,-1.4081690688991E-16));
#126574=DIRECTION('center_axis',(-1.4081690688991E-16,-6.98296267768627E-15,
1.));
#126575=DIRECTION('ref_axis',(-1.,7.97077743482043E-31,-1.4081690688991E-16));
#126576=DIRECTION('center_axis',(-1.4081690688991E-16,-6.98296267768627E-15,
1.));
#126577=DIRECTION('ref_axis',(-1.,7.97077743482043E-31,-1.4081690688991E-16));
#126578=DIRECTION('',(-0.809016994374955,0.587785252292463,3.99055920848342E-15));
#126579=DIRECTION('center_axis',(1.4081690688991E-16,6.98296267768627E-15,
-1.));
#126580=DIRECTION('ref_axis',(1.,-7.97077743482043E-31,1.4081690688991E-16));
#126581=DIRECTION('',(0.433019586648926,-0.249998457755604,-0.866022406579768));
#126582=DIRECTION('center_axis',(1.4081690688991E-16,6.98296267768627E-15,
-1.));
#126583=DIRECTION('ref_axis',(-1.,7.97577417048809E-31,-1.40816906889911E-16));
#126584=DIRECTION('',(-0.404509888559958,0.29389954297172,0.866022406579775));
#126585=DIRECTION('center_axis',(-1.4081690688991E-16,-6.98296267768627E-15,
1.));
#126586=DIRECTION('ref_axis',(-1.,9.83319205199467E-31,-1.40816906889911E-16));
#126587=DIRECTION('center_axis',(-1.4081690688991E-16,-6.98296267768627E-15,
1.));
#126588=DIRECTION('ref_axis',(-1.,7.98248735348668E-31,-1.4081690688991E-16));
#126589=DIRECTION('',(0.866025403784445,-0.499999999999989,-3.36953032019404E-15));
#126590=DIRECTION('center_axis',(1.4081690688991E-16,6.98296267768627E-15,
-1.));
#126591=DIRECTION('ref_axis',(-1.,7.98707387273907E-31,-1.4081690688991E-16));
#126592=DIRECTION('',(-0.809016994374955,0.587785252292463,3.99055920848342E-15));
#126593=DIRECTION('center_axis',(-1.4081690688991E-16,-6.98296267768627E-15,
1.));
#126594=DIRECTION('ref_axis',(-1.,7.99150043815584E-31,-1.4081690688991E-16));
#126595=DIRECTION('center_axis',(-1.4081690688991E-16,-6.98296267768627E-15,
1.));
#126596=DIRECTION('ref_axis',(1.,2.66453525910038E-14,1.40816906890097E-16));
#126597=DIRECTION('',(0.433014711050254,-0.250006503598669,0.866022521746654));
#126598=DIRECTION('center_axis',(-1.4081690688991E-16,-6.98296267768627E-15,
1.));
#126599=DIRECTION('ref_axis',(-1.,7.99858039355471E-31,-1.4081690688991E-16));
#126600=DIRECTION('center_axis',(-1.4081690688991E-16,-6.98296267768627E-15,
1.));
#126601=DIRECTION('ref_axis',(-1.,7.99858039355471E-31,-1.4081690688991E-16));
#126602=DIRECTION('center_axis',(-1.4081690688991E-16,-6.98296267768627E-15,
1.));
#126603=DIRECTION('ref_axis',(-1.,7.99858039355471E-31,-1.4081690688991E-16));
#126604=DIRECTION('',(-0.404515255718701,0.293891816351536,-0.866022521746651));
#126605=DIRECTION('center_axis',(-1.4081690688991E-16,-6.98296267768627E-15,
1.));
#126606=DIRECTION('ref_axis',(-1.,9.83319205199467E-31,-1.40816906889911E-16));
#126607=DIRECTION('',(0.866025403784445,-0.499999999999989,-3.36953032019404E-15));
#126608=DIRECTION('center_axis',(1.4081690688991E-16,6.98296267768627E-15,
-1.));
#126609=DIRECTION('ref_axis',(-1.,8.01265634860448E-31,-1.4081690688991E-16));
#126610=DIRECTION('',(-0.809016994374955,0.587785252292463,3.99055920848342E-15));
#126611=DIRECTION('center_axis',(-1.4081690688991E-16,-6.98296267768627E-15,
1.));
#126612=DIRECTION('ref_axis',(-1.,8.32577322149061E-31,-1.39145123902276E-16));
#126613=DIRECTION('center_axis',(0.500926582476573,0.865489779781651,-7.86457212410024E-6));
#126614=DIRECTION('ref_axis',(5.20726760504278E-6,6.07299298703026E-6,0.999999999968002));
#126615=DIRECTION('center_axis',(-0.586919060371635,-0.809645611678731,
-7.86457216103576E-6));
#126616=DIRECTION('ref_axis',(-0.686618216540855,0.49773029711256,0.529924500330469));
#126617=DIRECTION('center_axis',(-1.4081690688991E-16,-6.98296267768627E-15,
1.));
#126618=DIRECTION('ref_axis',(-1.,8.07722881720021E-31,-1.42096112075504E-16));
#126619=DIRECTION('center_axis',(0.500887108754422,0.865512625088838,9.77059208168159E-6));
#126620=DIRECTION('ref_axis',(0.757015822392275,-0.438092662174016,-0.484769908303961));
#126621=DIRECTION('center_axis',(-0.586955986038978,-0.809618842639886,
9.77052194850957E-6));
#126622=DIRECTION('ref_axis',(0.708129726178852,-0.513384442288873,-0.484756336026264));
#126623=DIRECTION('center_axis',(-1.4081690688991E-16,-6.98296267768627E-15,
1.));
#126624=DIRECTION('ref_axis',(-1.,8.24049048117772E-31,-1.37719829560012E-16));
#126625=DIRECTION('center_axis',(-0.497748107605237,-0.867321636444941,
-1.81624800435674E-5));
#126626=DIRECTION('ref_axis',(0.750441041150478,-0.4306818810425,0.501349539840898));
#126627=DIRECTION('center_axis',(0.589885332530148,0.807487024129206,-1.81316451594575E-5));
#126628=DIRECTION('ref_axis',(0.700081622910561,-0.511412360642604,0.498340364254066));
#126629=DIRECTION('center_axis',(-1.4081690688991E-16,-6.98296267768627E-15,
1.));
#126630=DIRECTION('ref_axis',(-1.,8.26087817385229E-31,-1.38060560438432E-16));
#126631=DIRECTION('center_axis',(-0.497736388324913,-0.867328361922543,
-1.84940447271398E-5));
#126632=DIRECTION('ref_axis',(0.751962698441535,-0.43152051494869,-0.498339387697724));
#126633=DIRECTION('center_axis',(0.589896242833519,0.807479053813593,-1.85257084974504E-5));
#126634=DIRECTION('ref_axis',(0.698662091932916,-0.510412535075953,-0.501348506862502));
#126635=DIRECTION('center_axis',(-1.4081690688991E-16,-6.98296267768627E-15,
1.));
#126636=DIRECTION('ref_axis',(-1.,9.83319205199467E-31,-1.40816906889911E-16));
#126637=DIRECTION('center_axis',(-1.4081690688991E-16,-6.98296267768627E-15,
1.));
#126638=DIRECTION('ref_axis',(-1.,8.46073526001725E-31,-1.4081690688991E-16));
#126639=DIRECTION('',(0.809016994374955,-0.587785252292463,-3.99055920848342E-15));
#126640=DIRECTION('center_axis',(-1.4081690688991E-16,-6.98296267768627E-15,
1.));
#126641=DIRECTION('ref_axis',(-1.,7.97077743482043E-31,-1.4081690688991E-16));
#126642=DIRECTION('center_axis',(-1.4081690688991E-16,-6.98296267768627E-15,
1.));
#126643=DIRECTION('ref_axis',(-1.,7.97077743482043E-31,-1.4081690688991E-16));
#126644=DIRECTION('center_axis',(-1.4081690688991E-16,-6.98296267768627E-15,
1.));
#126645=DIRECTION('ref_axis',(-1.,7.97077743482043E-31,-1.4081690688991E-16));
#126646=DIRECTION('',(-0.743144825477402,0.66913060635885,4.56786669500646E-15));
#126647=DIRECTION('center_axis',(1.4081690688991E-16,6.98296267768627E-15,
-1.));
#126648=DIRECTION('ref_axis',(1.,-7.97077743482043E-31,1.4081690688991E-16));
#126649=DIRECTION('',(0.404515505437167,-0.293891812003452,-0.866022406579784));
#126650=DIRECTION('center_axis',(1.4081690688991E-16,6.98296267768627E-15,
-1.));
#126651=DIRECTION('ref_axis',(-1.,7.97577417048809E-31,-1.40816906889911E-16));
#126652=DIRECTION('',(-0.371573073483921,0.33457232755186,0.866022406579786));
#126653=DIRECTION('center_axis',(-1.4081690688991E-16,-6.98296267768627E-15,
1.));
#126654=DIRECTION('ref_axis',(-1.,9.83319205199467E-31,-1.40816906889911E-16));
#126655=DIRECTION('center_axis',(-1.4081690688991E-16,-6.98296267768627E-15,
1.));
#126656=DIRECTION('ref_axis',(-1.,7.98248735348668E-31,-1.4081690688991E-16));
#126657=DIRECTION('',(0.809016994374955,-0.587785252292463,-3.99055920848342E-15));
#126658=DIRECTION('center_axis',(1.4081690688991E-16,6.98296267768627E-15,
-1.));
#126659=DIRECTION('ref_axis',(-1.,7.98707387273907E-31,-1.4081690688991E-16));
#126660=DIRECTION('',(-0.743144825477402,0.66913060635885,4.56786669500646E-15));
#126661=DIRECTION('center_axis',(-1.4081690688991E-16,-6.98296267768627E-15,
1.));
#126662=DIRECTION('ref_axis',(-1.,7.99150043815584E-31,-1.4081690688991E-16));
#126663=DIRECTION('center_axis',(-1.4081690688991E-16,-6.98296267768627E-15,
1.));
#126664=DIRECTION('ref_axis',(1.,-1.95399252334028E-14,1.40816906889774E-16));
#126665=DIRECTION('',(0.404509815527881,-0.293899304131704,0.866022521746692));
#126666=DIRECTION('center_axis',(-1.4081690688991E-16,-6.98296267768627E-15,
1.));
#126667=DIRECTION('ref_axis',(-1.,7.99858039355471E-31,-1.4081690688991E-16));
#126668=DIRECTION('center_axis',(-1.4081690688991E-16,-6.98296267768627E-15,
1.));
#126669=DIRECTION('ref_axis',(-1.,7.99858039355471E-31,-1.4081690688991E-16));
#126670=DIRECTION('center_axis',(-1.4081690688991E-16,-6.98296267768627E-15,
1.));
#126671=DIRECTION('ref_axis',(-1.,7.99858039355471E-31,-1.4081690688991E-16));
#126672=DIRECTION('',(-0.371579218892574,0.334565204279747,-0.866022521746655));
#126673=DIRECTION('center_axis',(-1.4081690688991E-16,-6.98296267768627E-15,
1.));
#126674=DIRECTION('ref_axis',(-1.,9.83319205199467E-31,-1.40816906889911E-16));
#126675=DIRECTION('',(0.809016994374955,-0.587785252292463,-3.99055920848342E-15));
#126676=DIRECTION('center_axis',(1.4081690688991E-16,6.98296267768627E-15,
-1.));
#126677=DIRECTION('ref_axis',(-1.,8.01265634860448E-31,-1.4081690688991E-16));
#126678=DIRECTION('',(-0.743144825477402,0.66913060635885,4.56786669500646E-15));
#126679=DIRECTION('center_axis',(-1.4081690688991E-16,-6.98296267768627E-15,
1.));
#126680=DIRECTION('ref_axis',(-1.,8.32577322149061E-31,-1.39145123902276E-16));
#126681=DIRECTION('center_axis',(0.588650770899369,0.808387450334137,-7.86457205642189E-6));
#126682=DIRECTION('ref_axis',(5.81354222511562E-6,5.49541676348314E-6,0.999999999968002));
#126683=DIRECTION('center_axis',(-0.668334867928742,-0.743860540860193,
-7.86457217696032E-6));
#126684=DIRECTION('ref_axis',(-0.63082986702967,0.566774825493184,0.529924500330471));
#126685=DIRECTION('center_axis',(-1.4081690688991E-16,-6.98296267768627E-15,
1.));
#126686=DIRECTION('ref_axis',(-1.,8.07722881720021E-31,-1.42096112075504E-16));
#126687=DIRECTION('center_axis',(0.588613901402471,0.808414296620426,9.77059026348027E-6));
#126688=DIRECTION('ref_axis',(0.707075657763682,-0.514822445316384,-0.484769908303429));
#126689=DIRECTION('center_axis',(-0.66836879318871,-0.743830058680075,9.77051759200369E-6));
#126690=DIRECTION('ref_axis',(0.650587230627419,-0.584591780668772,-0.484756336027762));
#126691=DIRECTION('center_axis',(-1.4081690688991E-16,-6.98296267768627E-15,
1.));
#126692=DIRECTION('ref_axis',(-1.,8.24049048117772E-31,-1.37719829560012E-16));
#126693=DIRECTION('center_axis',(-0.585681189207855,-0.810541512988815,
-1.81624800237498E-5));
#126694=DIRECTION('ref_axis',(0.701311531421822,-0.506765009437568,0.501349539846722));
#126695=DIRECTION('center_axis',(0.671059256698578,0.7414037184088,-1.81316451876482E-5));
#126696=DIRECTION('ref_axis',(0.642789354375964,-0.581789246426184,0.498340364252971));
#126697=DIRECTION('center_axis',(-1.4081690688991E-16,-6.98296267768627E-15,
1.));
#126698=DIRECTION('ref_axis',(-1.,8.26087817385229E-31,-1.38060560438432E-16));
#126699=DIRECTION('center_axis',(-0.585670237138178,-0.810549426616589,
-1.84940603684897E-5));
#126700=DIRECTION('ref_axis',(0.70273719180265,-0.507758105718623,-0.498339387701155));
#126701=DIRECTION('center_axis',(0.671069274107353,0.741394651319949,-1.85257130833385E-5));
#126702=DIRECTION('ref_axis',(0.641482109969085,-0.580646516618343,-0.501348506857849));
#126703=DIRECTION('center_axis',(-1.4081690688991E-16,-6.98296267768627E-15,
1.));
#126704=DIRECTION('ref_axis',(-1.,9.83319205199467E-31,-1.40816906889911E-16));
#126705=DIRECTION('center_axis',(-1.4081690688991E-16,-6.98296267768627E-15,
1.));
#126706=DIRECTION('ref_axis',(-1.,8.46073526001725E-31,-1.4081690688991E-16));
#126707=DIRECTION('',(0.743144825477402,-0.66913060635885,-4.56786669500646E-15));
#126708=DIRECTION('center_axis',(-1.4081690688991E-16,-6.98296267768627E-15,
1.));
#126709=DIRECTION('ref_axis',(-1.,7.97077743482043E-31,-1.4081690688991E-16));
#126710=DIRECTION('center_axis',(-1.4081690688991E-16,-6.98296267768627E-15,
1.));
#126711=DIRECTION('ref_axis',(-1.,7.97077743482043E-31,-1.4081690688991E-16));
#126712=DIRECTION('center_axis',(-1.4081690688991E-16,-6.98296267768627E-15,
1.));
#126713=DIRECTION('ref_axis',(-1.,7.97077743482043E-31,-1.4081690688991E-16));
#126714=DIRECTION('',(-0.669130606358867,0.743144825477386,5.09512767813144E-15));
#126715=DIRECTION('center_axis',(1.4081690688991E-16,6.98296267768627E-15,
-1.));
#126716=DIRECTION('ref_axis',(1.,-7.97077743482043E-31,1.4081690688991E-16));
#126717=DIRECTION('',(0.371579467697567,-0.33456522605815,-0.86602240657979));
#126718=DIRECTION('center_axis',(1.4081690688991E-16,6.98296267768627E-15,
-1.));
#126719=DIRECTION('ref_axis',(-1.,7.97577417048809E-31,-1.40816906889911E-16));
#126720=DIRECTION('',(-0.334565226058174,0.371579467697563,0.866022406579783));
#126721=DIRECTION('center_axis',(-1.4081690688991E-16,-6.98296267768627E-15,
1.));
#126722=DIRECTION('ref_axis',(-1.,9.83319205199467E-31,-1.40816906889911E-16));
#126723=DIRECTION('center_axis',(-1.4081690688991E-16,-6.98296267768627E-15,
1.));
#126724=DIRECTION('ref_axis',(-1.,7.98248735348668E-31,-1.4081690688991E-16));
#126725=DIRECTION('',(0.743144825477402,-0.66913060635885,-4.56786669500646E-15));
#126726=DIRECTION('center_axis',(1.4081690688991E-16,6.98296267768627E-15,
-1.));
#126727=DIRECTION('ref_axis',(-1.,7.98707387273907E-31,-1.4081690688991E-16));
#126728=DIRECTION('',(-0.669130606358867,0.743144825477386,5.09512767813144E-15));
#126729=DIRECTION('center_axis',(-1.4081690688991E-16,-6.98296267768627E-15,
1.));
#126730=DIRECTION('ref_axis',(-1.,7.99150043815584E-31,-1.4081690688991E-16));
#126731=DIRECTION('center_axis',(-1.4081690688991E-16,-6.98296267768627E-15,
1.));
#126732=DIRECTION('ref_axis',(1.,3.19744231092045E-14,1.40816906890134E-16));
#126733=DIRECTION('',(0.3715730258176,-0.334572082386297,0.866022521746663));
#126734=DIRECTION('center_axis',(-1.4081690688991E-16,-6.98296267768627E-15,
1.));
#126735=DIRECTION('ref_axis',(-1.,7.99858039355471E-31,-1.4081690688991E-16));
#126736=DIRECTION('center_axis',(-1.4081690688991E-16,-6.98296267768627E-15,
1.));
#126737=DIRECTION('ref_axis',(-1.,7.99858039355471E-31,-1.4081690688991E-16));
#126738=DIRECTION('center_axis',(-1.4081690688991E-16,-6.98296267768627E-15,
1.));
#126739=DIRECTION('ref_axis',(-1.,7.99858039355471E-31,-1.4081690688991E-16));
#126740=DIRECTION('',(-0.334572082386318,0.371573025817621,-0.866022521746647));
#126741=DIRECTION('center_axis',(-1.4081690688991E-16,-6.98296267768627E-15,
1.));
#126742=DIRECTION('ref_axis',(-1.,9.83319205199467E-31,-1.40816906889911E-16));
#126743=DIRECTION('',(0.743144825477402,-0.66913060635885,-4.56786669500646E-15));
#126744=DIRECTION('center_axis',(1.4081690688991E-16,6.98296267768627E-15,
-1.));
#126745=DIRECTION('ref_axis',(-1.,8.01265634860448E-31,-1.4081690688991E-16));
#126746=DIRECTION('',(-0.669130606358867,0.743144825477386,5.09512767813144E-15));
#126747=DIRECTION('center_axis',(-1.4081690688991E-16,-6.98296267768627E-15,
1.));
#126748=DIRECTION('ref_axis',(-1.,8.32577322149061E-31,-1.39145123902276E-16));
#126749=DIRECTION('center_axis',(0.669925578293193,0.742428258814735,-7.86457219354815E-6));
#126750=DIRECTION('ref_axis',(6.35612258761182E-6,4.85763177036266E-6,0.999999999968002));
#126751=DIRECTION('center_axis',(-0.742428258814788,-0.669925578293134,
-7.86457211237817E-6));
#126752=DIRECTION('ref_axis',(-0.568130013485616,0.62960965028049,0.529924500330484));
#126753=DIRECTION('center_axis',(-1.4081690688991E-16,-6.98296267768627E-15,
1.));
#126754=DIRECTION('ref_axis',(-1.,8.07722881720021E-31,-1.42096112075504E-16));
#126755=DIRECTION('center_axis',(0.669891716967477,0.742458811950469,9.77057870806457E-6));
#126756=DIRECTION('ref_axis',(0.64938862426354,-0.585911726014409,-0.484769908302819));
#126757=DIRECTION('center_axis',(-0.742458811969724,-0.669891716946137,
9.77052681118192E-6));
#126758=DIRECTION('ref_axis',(0.585916765233986,-0.649394209166681,-0.484756336027208));
#126759=DIRECTION('center_axis',(-1.4081690688991E-16,-6.98296267768627E-15,
1.));
#126760=DIRECTION('ref_axis',(-1.,8.24049048117772E-31,-1.37719829560012E-16));
#126761=DIRECTION('center_axis',(-0.667197425139981,-0.744880927099563,
-1.81624800116486E-5));
#126762=DIRECTION('ref_axis',(0.6444983057982,-0.577295914343043,0.501349539848278));
#126763=DIRECTION('center_axis',(0.744880915222603,0.667197438400643,-1.8131645392542E-5));
#126764=DIRECTION('ref_axis',(0.578454551163162,-0.645791927479786,0.498340364249744));
#126765=DIRECTION('center_axis',(-1.4081690688991E-16,-6.98296267768627E-15,
1.));
#126766=DIRECTION('ref_axis',(-1.,8.26087817385229E-31,-1.38060560438432E-16));
#126767=DIRECTION('center_axis',(-0.667187360273293,-0.744889942172348,
-1.84940770019934E-5));
#126768=DIRECTION('ref_axis',(0.645812349433761,-0.578432592427061,-0.498339387703757));
#126769=DIRECTION('center_axis',(0.744889929987161,0.667187373876725,-1.85257100377501E-5));
#126770=DIRECTION('ref_axis',(0.577273915765722,-0.64451881341307,-0.50134850686236));
#126771=DIRECTION('center_axis',(-1.4081690688991E-16,-6.98296267768627E-15,
1.));
#126772=DIRECTION('ref_axis',(-1.,9.83319205199467E-31,-1.40816906889911E-16));
#126773=DIRECTION('center_axis',(-1.4081690688991E-16,-6.98296267768627E-15,
1.));
#126774=DIRECTION('ref_axis',(-1.,8.46073526001725E-31,-1.4081690688991E-16));
#126775=DIRECTION('',(0.669130606358867,-0.743144825477386,-5.09512767813144E-15));
#126776=DIRECTION('center_axis',(-1.4081690688991E-16,-6.98296267768627E-15,
1.));
#126777=DIRECTION('ref_axis',(-1.,7.97077743482043E-31,-1.4081690688991E-16));
#126778=DIRECTION('center_axis',(-1.4081690688991E-16,-6.98296267768627E-15,
1.));
#126779=DIRECTION('ref_axis',(-1.,7.97077743482043E-31,-1.4081690688991E-16));
#126780=DIRECTION('center_axis',(-1.4081690688991E-16,-6.98296267768627E-15,
1.));
#126781=DIRECTION('ref_axis',(-1.,7.97077743482043E-31,-1.4081690688991E-16));
#126782=DIRECTION('',(-0.587785252292482,0.809016994374941,5.5665653761908E-15));
#126783=DIRECTION('center_axis',(1.4081690688991E-16,6.98296267768627E-15,
-1.));
#126784=DIRECTION('ref_axis',(1.,-7.97077743482043E-31,1.4081690688991E-16));
#126785=DIRECTION('',(0.334572327551888,-0.371573073483894,-0.866022406579786));
#126786=DIRECTION('center_axis',(1.4081690688991E-16,6.98296267768627E-15,
-1.));
#126787=DIRECTION('ref_axis',(-1.,-1.86517468137026E-14,-1.40816906890041E-16));
#126788=DIRECTION('',(-0.29389181200343,0.404515505437148,0.8660224065798));
#126789=DIRECTION('center_axis',(-1.4081690688991E-16,-6.98296267768627E-15,
1.));
#126790=DIRECTION('ref_axis',(-1.,9.83319205199467E-31,-1.40816906889911E-16));
#126791=DIRECTION('center_axis',(-1.4081690688991E-16,-6.98296267768627E-15,
1.));
#126792=DIRECTION('ref_axis',(-1.,7.98248735348668E-31,-1.4081690688991E-16));
#126793=DIRECTION('',(0.669130606358867,-0.743144825477386,-5.09512767813144E-15));
#126794=DIRECTION('center_axis',(1.4081690688991E-16,6.98296267768627E-15,
-1.));
#126795=DIRECTION('ref_axis',(-1.,-1.86517468137026E-14,-1.40816906890041E-16));
#126796=DIRECTION('',(-0.587785252292482,0.809016994374941,5.5665653761908E-15));
#126797=DIRECTION('center_axis',(-1.4081690688991E-16,-6.98296267768627E-15,
1.));
#126798=DIRECTION('ref_axis',(-1.,7.99150043815584E-31,-1.4081690688991E-16));
#126799=DIRECTION('center_axis',(-1.4081690688991E-16,-6.98296267768627E-15,
1.));
#126800=DIRECTION('ref_axis',(1.,2.57571741713036E-14,1.4081690689009E-16));
#126801=DIRECTION('',(0.33456520427975,-0.371579218892551,0.866022521746664));
#126802=DIRECTION('center_axis',(-1.4081690688991E-16,-6.98296267768627E-15,
1.));
#126803=DIRECTION('ref_axis',(-1.,7.99858039355471E-31,-1.4081690688991E-16));
#126804=DIRECTION('center_axis',(-1.4081690688991E-16,-6.98296267768627E-15,
1.));
#126805=DIRECTION('ref_axis',(-1.,7.99858039355471E-31,-1.4081690688991E-16));
#126806=DIRECTION('center_axis',(-1.4081690688991E-16,-6.98296267768627E-15,
1.));
#126807=DIRECTION('ref_axis',(-1.,7.99858039355471E-31,-1.4081690688991E-16));
#126808=DIRECTION('',(-0.29389930413172,0.404509815527947,-0.866022521746656));
#126809=DIRECTION('center_axis',(-1.4081690688991E-16,-6.98296267768627E-15,
1.));
#126810=DIRECTION('ref_axis',(-1.,9.83319205199467E-31,-1.40816906889911E-16));
#126811=DIRECTION('',(0.669130606358867,-0.743144825477386,-5.09512767813144E-15));
#126812=DIRECTION('center_axis',(1.4081690688991E-16,6.98296267768627E-15,
-1.));
#126813=DIRECTION('ref_axis',(-1.,8.01265634860448E-31,-1.4081690688991E-16));
#126814=DIRECTION('',(-0.587785252292482,0.809016994374941,5.5665653761908E-15));
#126815=DIRECTION('center_axis',(-1.4081690688991E-16,-6.98296267768627E-15,
1.));
#126816=DIRECTION('ref_axis',(-1.,8.32577322149061E-31,-1.39145123902276E-16));
#126817=DIRECTION('center_axis',(0.74386054086017,0.668334867928768,-7.86457204182447E-6));
#126818=DIRECTION('ref_axis',(6.82906376097728E-6,4.16662531338862E-6,0.999999999968002));
#126819=DIRECTION('center_axis',(-0.808387450334084,-0.588650770899442,
-7.86457221610675E-6));
#126820=DIRECTION('ref_axis',(-0.49920560862511,0.685546339984938,0.529924500330461));
#126821=DIRECTION('center_axis',(-1.4081690688991E-16,-6.98296267768627E-15,
1.));
#126822=DIRECTION('ref_axis',(-1.,8.07722881720021E-31,-1.42096112075504E-16));
#126823=DIRECTION('center_axis',(0.743830058706459,0.668368793159347,9.77058883205476E-6));
#126824=DIRECTION('ref_axis',(0.58458675310207,-0.650581635231749,-0.484769908303684));
#126825=DIRECTION('center_axis',(-0.808414296645164,-0.588613901368497,
9.77051445187888E-6));
#126826=DIRECTION('ref_axis',(0.51482687315013,-0.707081738815272,-0.484756336025051));
#126827=DIRECTION('center_axis',(-1.4081690688991E-16,-6.98296267768627E-15,
1.));
#126828=DIRECTION('ref_axis',(-1.,8.24049048117772E-31,-1.37719829560012E-16));
#126829=DIRECTION('center_axis',(-0.741403706462227,-0.671059269896628,
-1.81624797328866E-5));
#126830=DIRECTION('ref_axis',(0.580623821869545,-0.641501844407148,0.501349539842046));
#126831=DIRECTION('center_axis',(0.810541502562919,0.585681203637515,-1.81316451185357E-5));
#126832=DIRECTION('ref_axis',(0.507782078836558,-0.702719177033379,0.498340364251134));
#126833=DIRECTION('center_axis',(-1.4081690688991E-16,-6.98296267768627E-15,
1.));
#126834=DIRECTION('ref_axis',(-1.,8.26087817385229E-31,-1.38060560438432E-16));
#126835=DIRECTION('center_axis',(-0.74139463905899,-0.671069287654084,-1.84940651197545E-5));
#126836=DIRECTION('ref_axis',(0.581811851821589,-0.642769650609858,-0.498339387701608));
#126837=DIRECTION('center_axis',(0.810549415920134,0.585670251940739,-1.85256933039895E-5));
#126838=DIRECTION('ref_axis',(0.506740987741753,-0.701329627216764,-0.501348506859757));
#126839=DIRECTION('center_axis',(-1.4081690688991E-16,-6.98296267768627E-15,
1.));
#126840=DIRECTION('ref_axis',(-1.,9.83319205199467E-31,-1.40816906889911E-16));
#126841=DIRECTION('center_axis',(-1.4081690688991E-16,-6.98296267768627E-15,
1.));
#126842=DIRECTION('ref_axis',(-1.,8.46073526001725E-31,-1.4081690688991E-16));
#126843=DIRECTION('',(0.587785252292482,-0.809016994374941,-5.5665653761908E-15));
#126844=DIRECTION('center_axis',(-1.4081690688991E-16,-6.98296267768627E-15,
1.));
#126845=DIRECTION('ref_axis',(-1.,7.97077743482043E-31,-1.4081690688991E-16));
#126846=DIRECTION('center_axis',(-1.4081690688991E-16,-6.98296267768627E-15,
1.));
#126847=DIRECTION('ref_axis',(-1.,7.97077743482043E-31,-1.4081690688991E-16));
#126848=DIRECTION('center_axis',(-1.4081690688991E-16,-6.98296267768627E-15,
1.));
#126849=DIRECTION('ref_axis',(-1.,7.97077743482043E-31,-1.4081690688991E-16));
#126850=DIRECTION('',(-0.50000000000001,0.866025403784433,5.97701461910992E-15));
#126851=DIRECTION('center_axis',(1.4081690688991E-16,6.98296267768627E-15,
-1.));
#126852=DIRECTION('ref_axis',(1.,-7.97077743482043E-31,1.4081690688991E-16));
#126853=DIRECTION('',(0.293899542971754,-0.404509888559887,-0.866022406579796));
#126854=DIRECTION('center_axis',(1.4081690688991E-16,6.98296267768627E-15,
-1.));
#126855=DIRECTION('ref_axis',(-1.,1.95399252334028E-14,-1.40816906889774E-16));
#126856=DIRECTION('',(-0.24999845775561,0.433019586648882,0.866022406579788));
#126857=DIRECTION('center_axis',(-1.4081690688991E-16,-6.98296267768627E-15,
1.));
#126858=DIRECTION('ref_axis',(-1.,9.83319205199467E-31,-1.40816906889911E-16));
#126859=DIRECTION('center_axis',(-1.4081690688991E-16,-6.98296267768627E-15,
1.));
#126860=DIRECTION('ref_axis',(-1.,7.98248735348668E-31,-1.4081690688991E-16));
#126861=DIRECTION('',(0.587785252292482,-0.809016994374941,-5.5665653761908E-15));
#126862=DIRECTION('center_axis',(1.4081690688991E-16,6.98296267768627E-15,
-1.));
#126863=DIRECTION('ref_axis',(-1.,1.86517468137026E-14,-1.4081690688978E-16));
#126864=DIRECTION('',(-0.50000000000001,0.866025403784433,5.97701461910992E-15));
#126865=DIRECTION('center_axis',(-1.4081690688991E-16,-6.98296267768627E-15,
1.));
#126866=DIRECTION('ref_axis',(-1.,7.99150043815584E-31,-1.4081690688991E-16));
#126867=DIRECTION('center_axis',(-1.4081690688991E-16,-6.98296267768627E-15,
1.));
#126868=DIRECTION('ref_axis',(1.,-1.24344978758018E-14,1.40816906889824E-16));
#126869=DIRECTION('',(0.293891816351536,-0.404515255718701,0.866022521746651));
#126870=DIRECTION('center_axis',(-1.4081690688991E-16,-6.98296267768627E-15,
1.));
#126871=DIRECTION('ref_axis',(-1.,7.99858039355471E-31,-1.4081690688991E-16));
#126872=DIRECTION('center_axis',(-1.4081690688991E-16,-6.98296267768627E-15,
1.));
#126873=DIRECTION('ref_axis',(-1.,7.99858039355471E-31,-1.4081690688991E-16));
#126874=DIRECTION('center_axis',(-1.4081690688991E-16,-6.98296267768627E-15,
1.));
#126875=DIRECTION('ref_axis',(-1.,7.99858039355471E-31,-1.4081690688991E-16));
#126876=DIRECTION('',(-0.250006503598685,0.433014711050231,-0.866022521746661));
#126877=DIRECTION('center_axis',(-1.4081690688991E-16,-6.98296267768627E-15,
1.));
#126878=DIRECTION('ref_axis',(-1.,9.83319205199467E-31,-1.40816906889911E-16));
#126879=DIRECTION('',(0.587785252292482,-0.809016994374941,-5.5665653761908E-15));
#126880=DIRECTION('center_axis',(1.4081690688991E-16,6.98296267768627E-15,
-1.));
#126881=DIRECTION('ref_axis',(-1.,-1.95399252334028E-14,-1.40816906890047E-16));
#126882=DIRECTION('',(-0.50000000000001,0.866025403784433,5.97701461910992E-15));
#126883=DIRECTION('center_axis',(-1.4081690688991E-16,-6.98296267768627E-15,
1.));
#126884=DIRECTION('ref_axis',(-1.,8.32577322149061E-31,-1.39145123902276E-16));
#126885=DIRECTION('center_axis',(0.809645611678629,0.586919060371776,-7.86457187793608E-6));
#126886=DIRECTION('ref_axis',(7.22718427493033E-6,3.42996842081855E-6,0.999999999968002));
#126887=DIRECTION('center_axis',(-0.865489779781559,-0.50092658247673,-7.86457232116346E-6));
#126888=DIRECTION('ref_axis',(-0.424811802651054,0.733972040528688,0.529924500330486));
#126889=DIRECTION('center_axis',(-1.4081690688991E-16,-6.98296267768627E-15,
1.));
#126890=DIRECTION('ref_axis',(-1.,8.07722881720021E-31,-1.42096112075504E-16));
#126891=DIRECTION('center_axis',(0.809618842658828,0.586955986012849,9.77058027889881E-6));
#126892=DIRECTION('ref_axis',(0.513380027141257,-0.70812363591068,-0.484769908304012));
#126893=DIRECTION('center_axis',(-0.865512625108597,-0.500887108720281,
9.77052087483086E-6));
#126894=DIRECTION('ref_axis',(0.43809643010891,-0.757022332966292,-0.48475633602471));
#126895=DIRECTION('center_axis',(-1.4081690688991E-16,-6.98296267768627E-15,
1.));
#126896=DIRECTION('ref_axis',(-1.,8.24049048117772E-31,-1.37719829560012E-16));
#126897=DIRECTION('center_axis',(-0.807487013627711,-0.589885346904571,
-1.81624797236099E-5));
#126898=DIRECTION('ref_axis',(0.510387901842864,-0.698679346019309,0.501349539840688));
#126899=DIRECTION('center_axis',(0.867321627584552,0.497748123045508,-1.81316453750404E-5));
#126900=DIRECTION('ref_axis',(0.431546239794831,-0.751947288230892,0.498340364250329));
#126901=DIRECTION('center_axis',(-1.4081690688991E-16,-6.98296267768627E-15,
1.));
#126902=DIRECTION('ref_axis',(-1.,8.26087817385229E-31,-1.38060560438432E-16));
#126903=DIRECTION('center_axis',(-0.807479043037464,-0.589896257585408,
-1.84940653406147E-5));
#126904=DIRECTION('ref_axis',(0.511436901809794,-0.700064389993911,-0.49833938769643));
#126905=DIRECTION('center_axis',(0.867328352821041,0.497736404183517,-1.85257158465585E-5));
#126906=DIRECTION('ref_axis',(0.430656099411607,-0.750456526859266,-0.501348506863148));
#126907=DIRECTION('center_axis',(-1.4081690688991E-16,-6.98296267768627E-15,
1.));
#126908=DIRECTION('ref_axis',(-1.,9.83319205199467E-31,-1.40816906889911E-16));
#126909=DIRECTION('center_axis',(-1.4081690688991E-16,-6.98296267768627E-15,
1.));
#126910=DIRECTION('ref_axis',(-1.,8.46073526001725E-31,-1.4081690688991E-16));
#126911=DIRECTION('',(0.50000000000001,-0.866025403784433,-5.97701461910992E-15));
#126912=DIRECTION('center_axis',(-1.4081690688991E-16,-6.98296267768627E-15,
1.));
#126913=DIRECTION('ref_axis',(-1.,7.97077743482043E-31,-1.4081690688991E-16));
#126914=DIRECTION('center_axis',(-1.4081690688991E-16,-6.98296267768627E-15,
1.));
#126915=DIRECTION('ref_axis',(-1.,7.97077743482043E-31,-1.4081690688991E-16));
#126916=DIRECTION('center_axis',(-1.4081690688991E-16,-6.98296267768627E-15,
1.));
#126917=DIRECTION('ref_axis',(-1.,7.97077743482043E-31,-1.4081690688991E-16));
#126918=DIRECTION('',(-0.40673664307581,0.913545457642596,6.32197843909135E-15));
#126919=DIRECTION('center_axis',(1.4081690688991E-16,6.98296267768627E-15,
-1.));
#126920=DIRECTION('ref_axis',(1.,-7.97077743482043E-31,1.4081690688991E-16));
#126921=DIRECTION('',(0.25000673349641,-0.433014808647711,-0.866022406579784));
#126922=DIRECTION('center_axis',(1.4081690688991E-16,6.98296267768627E-15,
-1.));
#126923=DIRECTION('ref_axis',(-1.,1.95399252334028E-14,-1.40816906889774E-16));
#126924=DIRECTION('',(-0.203366068089037,0.456779414654113,0.86602240657979));
#126925=DIRECTION('center_axis',(-1.4081690688991E-16,-6.98296267768627E-15,
1.));
#126926=DIRECTION('ref_axis',(-1.,9.83319205199467E-31,-1.40816906889911E-16));
#126927=DIRECTION('center_axis',(-1.4081690688991E-16,-6.98296267768627E-15,
1.));
#126928=DIRECTION('ref_axis',(-1.,7.98248735348668E-31,-1.4081690688991E-16));
#126929=DIRECTION('',(0.50000000000001,-0.866025403784433,-5.97701461910992E-15));
#126930=DIRECTION('center_axis',(1.4081690688991E-16,6.98296267768627E-15,
-1.));
#126931=DIRECTION('ref_axis',(-1.,2.04281036531029E-14,-1.40816906889768E-16));
#126932=DIRECTION('',(-0.40673664307581,0.913545457642596,6.32197843909135E-15));
#126933=DIRECTION('center_axis',(-1.4081690688991E-16,-6.98296267768627E-15,
1.));
#126934=DIRECTION('ref_axis',(-1.,7.99150043815584E-31,-1.4081690688991E-16));
#126935=DIRECTION('center_axis',(-1.4081690688991E-16,-6.98296267768627E-15,
1.));
#126936=DIRECTION('ref_axis',(1.,-1.24344978758018E-14,1.40816906889824E-16));
#126937=DIRECTION('',(0.249998488182559,-0.433019338752883,0.866022521746664));
#126938=DIRECTION('center_axis',(-1.4081690688991E-16,-6.98296267768627E-15,
1.));
#126939=DIRECTION('ref_axis',(-1.,7.99858039355471E-31,-1.4081690688991E-16));
#126940=DIRECTION('center_axis',(-1.4081690688991E-16,-6.98296267768627E-15,
1.));
#126941=DIRECTION('ref_axis',(-1.,7.99858039355471E-31,-1.4081690688991E-16));
#126942=DIRECTION('center_axis',(-1.4081690688991E-16,-6.98296267768627E-15,
1.));
#126943=DIRECTION('ref_axis',(-1.,7.99858039355471E-31,-1.4081690688991E-16));
#126944=DIRECTION('',(-0.203374579494996,0.456775406784117,-0.866022521746656));
#126945=DIRECTION('center_axis',(-1.4081690688991E-16,-6.98296267768627E-15,
1.));
#126946=DIRECTION('ref_axis',(-1.,9.83319205199467E-31,-1.40816906889911E-16));
#126947=DIRECTION('',(0.50000000000001,-0.866025403784433,-5.97701461910992E-15));
#126948=DIRECTION('center_axis',(1.4081690688991E-16,6.98296267768627E-15,
-1.));
#126949=DIRECTION('ref_axis',(-1.,-3.90798504668055E-14,-1.40816906890183E-16));
#126950=DIRECTION('',(-0.40673664307581,0.913545457642596,6.32197843909135E-15));
#126951=DIRECTION('center_axis',(-1.4081690688991E-16,-6.98296267768627E-15,
1.));
#126952=DIRECTION('ref_axis',(-1.,8.32577322149061E-31,-1.39145123902276E-16));
#126953=DIRECTION('center_axis',(0.866560035746456,0.499072844768427,-7.86457212100349E-6));
#126954=DIRECTION('ref_axis',(7.54612252965276E-6,2.65573237658703E-6,0.999999999968002));
#126955=DIRECTION('center_axis',(-0.913109622086429,-0.4077141375907,-7.86457242400786E-6));
#126956=DIRECTION('ref_axis',(-0.345763669669516,0.774356189802966,0.529924500330474));
#126957=DIRECTION('center_axis',(-1.4081690688991E-16,-6.98296267768627E-15,
1.));
#126958=DIRECTION('ref_axis',(-1.,8.07722881720021E-31,-1.42096112075504E-16));
#126959=DIRECTION('center_axis',(0.866537273150592,0.4991123662516,9.77058020237922E-6));
#126960=DIRECTION('ref_axis',(0.43654860217139,-0.757907285850219,-0.484769908304301));
#126961=DIRECTION('center_axis',(-0.913128216133684,-0.40767249208777,9.77051909676145E-6));
#126962=DIRECTION('ref_axis',(0.356566110901339,-0.798668832019219,-0.484756336026412));
#126963=DIRECTION('center_axis',(-1.4081690688991E-16,-6.98296267768627E-15,
1.));
#126964=DIRECTION('ref_axis',(-1.,8.24049048117772E-31,-1.37719829560012E-16));
#126965=DIRECTION('center_axis',(-0.864723324094283,-0.50224851661051,-1.8162479892997E-5));
#126966=DIRECTION('ref_axis',(0.434560065157101,-0.748201970507024,0.501349539842277));
#126967=DIRECTION('center_axis',(0.914599195355538,0.404361609857126,-1.81316451782619E-5));
#126968=DIRECTION('ref_axis',(0.350582289841583,-0.792936907580423,0.498340364255423));
#126969=DIRECTION('center_axis',(-1.4081690688991E-16,-6.98296267768627E-15,
1.));
#126970=DIRECTION('ref_axis',(-1.,8.26087817385229E-31,-1.38060560438432E-16));
#126971=DIRECTION('center_axis',(-0.864716537645637,-0.502260200673028,
-1.84940690499114E-5));
#126972=DIRECTION('ref_axis',(0.435458542073093,-0.749689077418544,-0.498339387701703));
#126973=DIRECTION('center_axis',(0.914604658798975,0.404349252206565,-1.85257025671403E-5));
#126974=DIRECTION('ref_axis',(0.349852852737875,-0.791361267753813,-0.501348506859498));
#126975=DIRECTION('center_axis',(-1.4081690688991E-16,-6.98296267768627E-15,
1.));
#126976=DIRECTION('ref_axis',(-1.,9.83319205199467E-31,-1.40816906889911E-16));
#126977=DIRECTION('center_axis',(-1.4081690688991E-16,-6.98296267768627E-15,
1.));
#126978=DIRECTION('ref_axis',(-1.,8.46073526001725E-31,-1.4081690688991E-16));
#126979=DIRECTION('',(0.40673664307581,-0.913545457642596,-6.32197843909135E-15));
#126980=DIRECTION('center_axis',(-1.4081690688991E-16,-6.98296267768627E-15,
1.));
#126981=DIRECTION('ref_axis',(-1.,7.97077743482043E-31,-1.4081690688991E-16));
#126982=DIRECTION('center_axis',(-1.4081690688991E-16,-6.98296267768627E-15,
1.));
#126983=DIRECTION('ref_axis',(-1.,7.97077743482043E-31,-1.4081690688991E-16));
#126984=DIRECTION('center_axis',(-1.4081690688991E-16,-6.98296267768627E-15,
1.));
#126985=DIRECTION('ref_axis',(-1.,7.97077743482043E-31,-1.4081690688991E-16));
#126986=DIRECTION('',(-0.309016994374957,0.95105651629515,6.59767734033506E-15));
#126987=DIRECTION('center_axis',(1.4081690688991E-16,6.98296267768627E-15,
-1.));
#126988=DIRECTION('ref_axis',(1.,-7.97077743482043E-31,1.4081690688991E-16));
#126989=DIRECTION('',(0.203374797931567,-0.456775527877799,-0.866022406579791));
#126990=DIRECTION('center_axis',(1.4081690688991E-16,6.98296267768627E-15,
-1.));
#126991=DIRECTION('ref_axis',(-1.,2.04281036531029E-14,-1.40816906889768E-16));
#126992=DIRECTION('',(-0.154505557223407,0.475534671805162,0.866022406579784));
#126993=DIRECTION('center_axis',(-1.4081690688991E-16,-6.98296267768627E-15,
1.));
#126994=DIRECTION('ref_axis',(-1.,9.83319205199467E-31,-1.40816906889911E-16));
#126995=DIRECTION('center_axis',(-1.4081690688991E-16,-6.98296267768627E-15,
1.));
#126996=DIRECTION('ref_axis',(-1.,7.98248735348668E-31,-1.4081690688991E-16));
#126997=DIRECTION('',(0.40673664307581,-0.913545457642596,-6.32197843909135E-15));
#126998=DIRECTION('center_axis',(1.4081690688991E-16,6.98296267768627E-15,
-1.));
#126999=DIRECTION('ref_axis',(-1.,7.98707387273907E-31,-1.4081690688991E-16));
#127000=DIRECTION('',(-0.309016994374957,0.95105651629515,6.59767734033506E-15));
#127001=DIRECTION('center_axis',(-1.4081690688991E-16,-6.98296267768627E-15,
1.));
#127002=DIRECTION('ref_axis',(-1.,7.99150043815584E-31,-1.4081690688991E-16));
#127003=DIRECTION('center_axis',(-1.4081690688991E-16,-6.98296267768627E-15,
1.));
#127004=DIRECTION('ref_axis',(1.,-1.24344978758018E-14,1.40816906889824E-16));
#127005=DIRECTION('',(0.203366124261494,-0.456779171296592,0.866022521746668));
#127006=DIRECTION('center_axis',(-1.4081690688991E-16,-6.98296267768627E-15,
1.));
#127007=DIRECTION('ref_axis',(-1.,7.99858039355471E-31,-1.4081690688991E-16));
#127008=DIRECTION('center_axis',(-1.4081690688991E-16,-6.98296267768627E-15,
1.));
#127009=DIRECTION('ref_axis',(-1.,7.99858039355471E-31,-1.4081690688991E-16));
#127010=DIRECTION('center_axis',(-1.4081690688991E-16,-6.98296267768627E-15,
1.));
#127011=DIRECTION('ref_axis',(-1.,7.99858039355471E-31,-1.4081690688991E-16));
#127012=DIRECTION('',(-0.154514440939479,0.47553157557488,-0.866022521746653));
#127013=DIRECTION('center_axis',(-1.4081690688991E-16,-6.98296267768627E-15,
1.));
#127014=DIRECTION('ref_axis',(-1.,9.83319205199467E-31,-1.40816906889911E-16));
#127015=DIRECTION('',(0.40673664307581,-0.913545457642596,-6.32197843909135E-15));
#127016=DIRECTION('center_axis',(1.4081690688991E-16,6.98296267768627E-15,
-1.));
#127017=DIRECTION('ref_axis',(-1.,8.01265634860448E-31,-1.4081690688991E-16));
#127018=DIRECTION('',(-0.309016994374957,0.95105651629515,6.59767734033506E-15));
#127019=DIRECTION('center_axis',(-1.4081690688991E-16,-6.98296267768627E-15,
1.));
#127020=DIRECTION('ref_axis',(-1.,8.32577322149061E-31,-1.39145123902276E-16));
#127021=DIRECTION('center_axis',(0.9139802467232,0.405758682640246,-7.86457197746387E-6));
#127022=DIRECTION('ref_axis',(7.78238356101367E-6,1.85239937195226E-6,0.999999999968001));
#127023=DIRECTION('center_axis',(-0.95072524429128,-0.310034691293467,-7.86457228400698E-6));
#127024=DIRECTION('ref_axis',(-0.262927277567181,0.806256330617373,0.52992450033049));
#127025=DIRECTION('center_axis',(-1.4081690688991E-16,-6.98296267768627E-15,
1.));
#127026=DIRECTION('ref_axis',(-1.,8.07722881720021E-31,-1.42096112075504E-16));
#127027=DIRECTION('center_axis',(0.913961739943914,0.405800366957978,9.77058357183956E-6));
#127028=DIRECTION('ref_axis',(0.354934259362539,-0.799387144963771,-0.48476990830438));
#127029=DIRECTION('center_axis',(-0.950739383337938,-0.309991330321888,
9.77051914909191E-6));
#127030=DIRECTION('ref_axis',(0.271129178766832,-0.831564948216754,-0.484756336027174));
#127031=DIRECTION('center_axis',(-1.4081690688991E-16,-6.98296267768627E-15,
1.));
#127032=DIRECTION('ref_axis',(-1.,8.24049048117772E-31,-1.37719829560012E-16));
#127033=DIRECTION('center_axis',(-0.912485544867141,-0.409108946466148,
-1.81624799228571E-5));
#127034=DIRECTION('ref_axis',(0.353971097460695,-0.789527137635747,0.501349539841392));
#127035=DIRECTION('center_axis',(0.951856222950113,0.306544826252847,-1.81316452973037E-5));
#127036=DIRECTION('ref_axis',(0.265777286958593,-0.825238944241564,0.498340364253187));
#127037=DIRECTION('center_axis',(-1.4081690688991E-16,-6.98296267768627E-15,
1.));
#127038=DIRECTION('ref_axis',(-1.,8.26087817385229E-31,-1.38060560438432E-16));
#127039=DIRECTION('center_axis',(-0.912480016910859,-0.409121275902793,
-1.84940621727514E-5));
#127040=DIRECTION('ref_axis',(0.354709207425047,-0.791100014429281,-0.498339387704691));
#127041=DIRECTION('center_axis',(0.951860364738416,0.30653196521219,-1.85257001811446E-5));
#127042=DIRECTION('ref_axis',(0.265216544997311,-0.823595688995009,-0.501348506857781));
#127043=DIRECTION('center_axis',(-1.4081690688991E-16,-6.98296267768627E-15,
1.));
#127044=DIRECTION('ref_axis',(-1.,9.83319205199467E-31,-1.40816906889911E-16));
#127045=DIRECTION('center_axis',(-1.4081690688991E-16,-6.98296267768627E-15,
1.));
#127046=DIRECTION('ref_axis',(-1.,8.46073526001725E-31,-1.4081690688991E-16));
#127047=DIRECTION('',(0.309016994374957,-0.95105651629515,-6.59767734033506E-15));
#127048=DIRECTION('center_axis',(-1.4081690688991E-16,-6.98296267768627E-15,
1.));
#127049=DIRECTION('ref_axis',(-1.,7.97077743482043E-31,-1.4081690688991E-16));
#127050=DIRECTION('center_axis',(-1.4081690688991E-16,-6.98296267768627E-15,
1.));
#127051=DIRECTION('ref_axis',(-1.,7.97077743482043E-31,-1.4081690688991E-16));
#127052=DIRECTION('center_axis',(-1.4081690688991E-16,-6.98296267768627E-15,
1.));
#127053=DIRECTION('ref_axis',(-1.,7.97077743482043E-31,-1.4081690688991E-16));
#127054=DIRECTION('',(-0.20791169081777,0.978147600733803,6.80109070798531E-15));
#127055=DIRECTION('center_axis',(1.4081690688991E-16,6.98296267768627E-15,
-1.));
#127056=DIRECTION('ref_axis',(1.,-7.97077743482043E-31,1.4081690688991E-16));
#127057=DIRECTION('',(0.154514645521721,-0.475531718838048,-0.866022406579777));
#127058=DIRECTION('center_axis',(1.4081690688991E-16,6.98296267768627E-15,
-1.));
#127059=DIRECTION('ref_axis',(-1.,-3.10862446895044E-14,-1.40816906890128E-16));
#127060=DIRECTION('',(-0.103952251140494,0.489079871579876,0.866022406579781));
#127061=DIRECTION('center_axis',(-1.4081690688991E-16,-6.98296267768627E-15,
1.));
#127062=DIRECTION('ref_axis',(-1.,9.83319205199467E-31,-1.40816906889911E-16));
#127063=DIRECTION('center_axis',(-1.4081690688991E-16,-6.98296267768627E-15,
1.));
#127064=DIRECTION('ref_axis',(-1.,7.98248735348668E-31,-1.4081690688991E-16));
#127065=DIRECTION('',(0.309016994374957,-0.95105651629515,-6.59767734033506E-15));
#127066=DIRECTION('center_axis',(1.4081690688991E-16,6.98296267768627E-15,
-1.));
#127067=DIRECTION('ref_axis',(-1.,-3.10862446895044E-14,-1.40816906890128E-16));
#127068=DIRECTION('',(-0.20791169081777,0.978147600733803,6.80109070798531E-15));
#127069=DIRECTION('center_axis',(-1.4081690688991E-16,-6.98296267768627E-15,
1.));
#127070=DIRECTION('ref_axis',(-1.,7.99150043815584E-31,-1.4081690688991E-16));
#127071=DIRECTION('center_axis',(-1.4081690688991E-16,-6.98296267768627E-15,
1.));
#127072=DIRECTION('ref_axis',(1.,3.5527136788005E-14,1.40816906890159E-16));
#127073=DIRECTION('',(0.154505638525959,-0.475534435652405,0.866022521746654));
#127074=DIRECTION('center_axis',(-1.4081690688991E-16,-6.98296267768627E-15,
1.));
#127075=DIRECTION('ref_axis',(-1.,7.99858039355471E-31,-1.4081690688991E-16));
#127076=DIRECTION('center_axis',(-1.4081690688991E-16,-6.98296267768627E-15,
1.));
#127077=DIRECTION('ref_axis',(-1.,7.99858039355471E-31,-1.4081690688991E-16));
#127078=DIRECTION('center_axis',(-1.4081690688991E-16,-6.98296267768627E-15,
1.));
#127079=DIRECTION('ref_axis',(-1.,7.99858039355471E-31,-1.4081690688991E-16));
#127080=DIRECTION('',(-0.103961409834819,0.48907772091222,-0.866022521746672));
#127081=DIRECTION('center_axis',(-1.4081690688991E-16,-6.98296267768627E-15,
1.));
#127082=DIRECTION('ref_axis',(-1.,9.83319205199467E-31,-1.40816906889911E-16));
#127083=DIRECTION('',(0.309016994374957,-0.95105651629515,-6.59767734033506E-15));
#127084=DIRECTION('center_axis',(1.4081690688991E-16,6.98296267768627E-15,
-1.));
#127085=DIRECTION('ref_axis',(-1.,8.01265634860448E-31,-1.4081690688991E-16));
#127086=DIRECTION('',(-0.20791169081777,0.978147600733803,6.80109070798531E-15));
#127087=DIRECTION('center_axis',(-1.4081690688991E-16,-6.98296267768627E-15,
1.));
#127088=DIRECTION('ref_axis',(-1.,8.32577322149061E-31,-1.39145123902276E-16));
#127089=DIRECTION('center_axis',(0.951386698854222,0.30799894347451,-7.86457202755924E-6));
#127090=DIRECTION('ref_axis',(7.93337935782266E-6,1.02877115701158E-6,0.999999999968001));
#127091=DIRECTION('center_axis',(-0.977924521767598,-0.208958440039553,
-7.86457224718168E-6));
#127092=DIRECTION('ref_axis',(-0.177210199190854,0.829322958353518,0.529924500330478));
#127093=DIRECTION('center_axis',(-1.4081690688991E-16,-6.98296267768627E-15,
1.));
#127094=DIRECTION('ref_axis',(-1.,8.07722881720021E-31,-1.42096112075504E-16));
#127095=DIRECTION('center_axis',(0.951372650654724,0.308042333926263,9.77058391111578E-6));
#127096=DIRECTION('ref_axis',(0.269431182533837,-0.832108751235939,-0.484769908301851));
#127097=DIRECTION('center_axis',(-0.97793405090397,-0.208913838668213,9.770513827856E-6));
#127098=DIRECTION('ref_axis',(0.182721698612625,-0.855350264826529,-0.48475633602595));
#127099=DIRECTION('center_axis',(-1.4081690688991E-16,-6.98296267768627E-15,
1.));
#127100=DIRECTION('ref_axis',(-1.,8.24049048117772E-31,-1.37719829560012E-16));
#127101=DIRECTION('center_axis',(-0.950250383060607,-0.311487093092626,
-1.81624797655766E-5));
#127102=DIRECTION('ref_axis',(0.269503948345924,-0.82220208022159,0.501349539847448));
#127103=DIRECTION('center_axis',(0.978684514577279,0.205369473383652,-1.81316451809006E-5));
#127104=DIRECTION('ref_axis',(0.178060372502512,-0.84849949033992,0.498340364246328));
#127105=DIRECTION('center_axis',(-1.4081690688991E-16,-6.98296267768627E-15,
1.));
#127106=DIRECTION('ref_axis',(-1.,8.26087817385229E-31,-1.38060560438432E-16));
#127107=DIRECTION('center_axis',(-0.950246174164118,-0.311499932816086,
-1.84940623667029E-5));
#127108=DIRECTION('ref_axis',(0.270073604474823,-0.823843494138777,-0.498339387697971));
#127109=DIRECTION('center_axis',(0.978687289330155,0.205356249869322,-1.85257125721377E-5));
#127110=DIRECTION('ref_axis',(0.177674469288529,-0.846806623514797,-0.501348506863748));
#127111=DIRECTION('center_axis',(-1.4081690688991E-16,-6.98296267768627E-15,
1.));
#127112=DIRECTION('ref_axis',(-1.,9.83319205199467E-31,-1.40816906889911E-16));
#127113=DIRECTION('center_axis',(-1.4081690688991E-16,-6.98296267768627E-15,
1.));
#127114=DIRECTION('ref_axis',(-1.,8.46073526001725E-31,-1.4081690688991E-16));
#127115=DIRECTION('',(0.20791169081777,-0.978147600733803,-6.80109070798531E-15));
#127116=DIRECTION('center_axis',(-1.4081690688991E-16,-6.98296267768627E-15,
1.));
#127117=DIRECTION('ref_axis',(-1.,7.97077743482043E-31,-1.4081690688991E-16));
#127118=DIRECTION('center_axis',(-1.4081690688991E-16,-6.98296267768627E-15,
1.));
#127119=DIRECTION('ref_axis',(-1.,7.97077743482043E-31,-1.4081690688991E-16));
#127120=DIRECTION('center_axis',(-1.4081690688991E-16,-6.98296267768627E-15,
1.));
#127121=DIRECTION('ref_axis',(-1.,7.97077743482043E-31,-1.4081690688991E-16));
#127122=DIRECTION('',(-0.104528463267664,0.994521895368272,6.92998990261914E-15));
#127123=DIRECTION('center_axis',(1.4081690688991E-16,6.98296267768627E-15,
-1.));
#127124=DIRECTION('ref_axis',(1.,-7.97077743482043E-31,1.4081690688991E-16));
#127125=DIRECTION('',(0.103961598321227,-0.48907788477527,-0.866022406579786));
#127126=DIRECTION('center_axis',(1.4081690688991E-16,6.98296267768627E-15,
-1.));
#127127=DIRECTION('ref_axis',(-1.,-3.19744231092045E-14,-1.40816906890134E-16));
#127128=DIRECTION('',(-0.052260022440647,0.497266609935019,0.866022406579782));
#127129=DIRECTION('center_axis',(-1.4081690688991E-16,-6.98296267768627E-15,
1.));
#127130=DIRECTION('ref_axis',(-1.,9.83319205199467E-31,-1.40816906889911E-16));
#127131=DIRECTION('center_axis',(-1.4081690688991E-16,-6.98296267768627E-15,
1.));
#127132=DIRECTION('ref_axis',(-1.,7.98248735348668E-31,-1.4081690688991E-16));
#127133=DIRECTION('',(0.20791169081777,-0.978147600733803,-6.80109070798531E-15));
#127134=DIRECTION('center_axis',(1.4081690688991E-16,6.98296267768627E-15,
-1.));
#127135=DIRECTION('ref_axis',(-1.,-3.19744231092045E-14,-1.40816906890134E-16));
#127136=DIRECTION('',(-0.104528463267664,0.994521895368272,6.92998990261914E-15));
#127137=DIRECTION('center_axis',(-1.4081690688991E-16,-6.98296267768627E-15,
1.));
#127138=DIRECTION('ref_axis',(-1.,7.99150043815584E-31,-1.4081690688991E-16));
#127139=DIRECTION('center_axis',(-1.4081690688991E-16,-6.98296267768627E-15,
1.));
#127140=DIRECTION('ref_axis',(1.,2.30926389122033E-14,1.40816906890072E-16));
#127141=DIRECTION('',(0.103952356682315,-0.489079645219204,0.866022521746664));
#127142=DIRECTION('center_axis',(-1.4081690688991E-16,-6.98296267768627E-15,
1.));
#127143=DIRECTION('ref_axis',(-1.,7.99858039355471E-31,-1.4081690688991E-16));
#127144=DIRECTION('center_axis',(-1.4081690688991E-16,-6.98296267768627E-15,
1.));
#127145=DIRECTION('ref_axis',(-1.,7.99858039355471E-31,-1.4081690688991E-16));
#127146=DIRECTION('center_axis',(-1.4081690688991E-16,-6.98296267768627E-15,
1.));
#127147=DIRECTION('ref_axis',(-1.,7.99858039355471E-31,-1.4081690688991E-16));
#127148=DIRECTION('',(-0.0522693557686642,0.497265428393217,-0.866022521746657));
#127149=DIRECTION('center_axis',(-1.4081690688991E-16,-6.98296267768627E-15,
1.));
#127150=DIRECTION('ref_axis',(-1.,9.83319205199467E-31,-1.40816906889911E-16));
#127151=DIRECTION('',(0.20791169081777,-0.978147600733803,-6.80109070798531E-15));
#127152=DIRECTION('center_axis',(1.4081690688991E-16,6.98296267768627E-15,
-1.));
#127153=DIRECTION('ref_axis',(-1.,1.06581410364015E-14,-1.40816906889836E-16));
#127154=DIRECTION('',(-0.104528463267664,0.994521895368272,6.92998990261914E-15));
#127155=DIRECTION('center_axis',(-1.4081690688991E-16,-6.98296267768627E-15,
1.));
#127156=DIRECTION('ref_axis',(-1.,8.32577322149061E-31,-1.39145123902276E-16));
#127157=DIRECTION('center_axis',(0.978369559222101,0.206864703431255,-7.86457189927893E-6));
#127158=DIRECTION('ref_axis',(7.99745522714731E-6,1.93871412098472E-7,0.999999999968002));
#127159=DIRECTION('center_axis',(-0.994409453539564,-0.105592796389219,
-7.86457226194514E-6));
#127160=DIRECTION('ref_axis',(-0.0895515687886142,0.843303350210933,0.529924500330486));
#127161=DIRECTION('center_axis',(-1.4081690688991E-16,-6.98296267768627E-15,
1.));
#127162=DIRECTION('ref_axis',(-1.,8.07722881720021E-31,-1.42096112075504E-16));
#127163=DIRECTION('center_axis',(0.978360123517625,0.206909324620987,9.77058623646806E-6));
#127164=DIRECTION('ref_axis',(0.180976161286346,-0.855713599896903,-0.484769908304488));
#127165=DIRECTION('center_axis',(-0.994414268361322,-0.105547443284781,
9.77051728312679E-6));
#127166=DIRECTION('ref_axis',(0.0923122812911233,-0.869764184939502,-0.484756336028063));
#127167=DIRECTION('center_axis',(-1.4081690688991E-16,-6.98296267768627E-15,
1.));
#127168=DIRECTION('ref_axis',(-1.,8.24049048117772E-31,-1.37719829560012E-16));
#127169=DIRECTION('center_axis',(-0.97760407920455,-0.210452521944378,-1.81624797492279E-5));
#127170=DIRECTION('ref_axis',(0.182084057577984,-0.845868804766651,0.501349539840793));
#127171=DIRECTION('center_axis',(0.99479013385986,0.10194404958763,-1.81316452521936E-5));
#127172=DIRECTION('ref_axis',(0.0883925913421765,-0.862463698454775,0.498340364252713));
#127173=DIRECTION('center_axis',(-1.4081690688991E-16,-6.98296267768627E-15,
1.));
#127174=DIRECTION('ref_axis',(-1.,8.26087817385229E-31,-1.38060560438432E-16));
#127175=DIRECTION('center_axis',(-0.97760123548189,-0.210465731277688,-1.84940665228558E-5));
#127176=DIRECTION('ref_axis',(0.182479018596661,-0.847560772126245,-0.498339387691523));
#127177=DIRECTION('center_axis',(0.994791511178768,0.101930608471943,-1.85257116465804E-5));
#127178=DIRECTION('ref_axis',(0.0881857549144703,-0.860739767464731,-0.501348506864164));
#127179=DIRECTION('center_axis',(-1.4081690688991E-16,-6.98296267768627E-15,
1.));
#127180=DIRECTION('ref_axis',(-1.,9.83319205199467E-31,-1.40816906889911E-16));
#127181=DIRECTION('center_axis',(-1.4081690688991E-16,-6.98296267768627E-15,
1.));
#127182=DIRECTION('ref_axis',(-1.,8.46073526001725E-31,-1.4081690688991E-16));
#127183=DIRECTION('',(0.104528463267664,-0.994521895368272,-6.92998990261914E-15));
#127184=DIRECTION('center_axis',(-1.4081690688991E-16,-6.98296267768627E-15,
1.));
#127185=DIRECTION('ref_axis',(-1.,7.97077743482043E-31,-1.4081690688991E-16));
#127186=DIRECTION('center_axis',(-1.4081690688991E-16,-6.98296267768627E-15,
1.));
#127187=DIRECTION('ref_axis',(-1.,7.97077743482043E-31,-1.4081690688991E-16));
#127188=DIRECTION('center_axis',(-1.4081690688991E-16,-6.98296267768627E-15,
1.));
#127189=DIRECTION('ref_axis',(-1.,7.97077743482043E-31,-1.4081690688991E-16));
#127190=DIRECTION('',(-1.04744440165294E-14,1.,6.98296267768627E-15));
#127191=DIRECTION('center_axis',(1.4081690688991E-16,6.98296267768627E-15,
-1.));
#127192=DIRECTION('ref_axis',(1.,-7.97077743482043E-31,1.4081690688991E-16));
#127193=DIRECTION('',(0.0522695260941978,-0.497265611060804,-0.866022406579768));
#127194=DIRECTION('center_axis',(1.4081690688991E-16,6.98296267768627E-15,
-1.));
#127195=DIRECTION('ref_axis',(-1.,1.06581410364015E-14,-1.40816906889836E-16));
#127196=DIRECTION('',(4.77800116018645E-6,0.500005191251989,0.866022406579779));
#127197=DIRECTION('center_axis',(-1.4081690688991E-16,-6.98296267768627E-15,
1.));
#127198=DIRECTION('ref_axis',(-1.,9.83319205199467E-31,-1.40816906889911E-16));
#127199=DIRECTION('center_axis',(-1.4081690688991E-16,-6.98296267768627E-15,
1.));
#127200=DIRECTION('ref_axis',(-1.,7.98248735348668E-31,-1.4081690688991E-16));
#127201=DIRECTION('',(0.104528463267664,-0.994521895368272,-6.92998990261914E-15));
#127202=DIRECTION('center_axis',(1.4081690688991E-16,6.98296267768627E-15,
-1.));
#127203=DIRECTION('ref_axis',(-1.,1.06581410364015E-14,-1.40816906889836E-16));
#127204=DIRECTION('',(-1.04744440165294E-14,1.,6.98296267768627E-15));
#127205=DIRECTION('center_axis',(-1.4081690688991E-16,-6.98296267768627E-15,
1.));
#127206=DIRECTION('ref_axis',(-1.,7.99150043815584E-31,-1.4081690688991E-16));
#127207=DIRECTION('center_axis',(-1.4081690688991E-16,-6.98296267768627E-15,
1.));
#127208=DIRECTION('ref_axis',(1.,-2.30926389122033E-14,1.40816906889749E-16));
#127209=DIRECTION('',(0.0522601510654366,-0.497266395846486,0.866022521746671));
#127210=DIRECTION('center_axis',(-1.4081690688991E-16,-6.98296267768627E-15,
1.));
#127211=DIRECTION('ref_axis',(-1.,7.99858039355471E-31,-1.4081690688991E-16));
#127212=DIRECTION('center_axis',(-1.4081690688991E-16,-6.98296267768627E-15,
1.));
#127213=DIRECTION('ref_axis',(-1.,7.99858039355471E-31,-1.4081690688991E-16));
#127214=DIRECTION('center_axis',(-1.4081690688991E-16,-6.98296267768627E-15,
1.));
#127215=DIRECTION('ref_axis',(-1.,7.99858039355471E-31,-1.4081690688991E-16));
#127216=DIRECTION('',(-4.62770265767274E-6,0.500004991781207,-0.866022521746669));
#127217=DIRECTION('center_axis',(-1.4081690688991E-16,-6.98296267768627E-15,
1.));
#127218=DIRECTION('ref_axis',(-1.,9.83319205199467E-31,-1.40816906889911E-16));
#127219=DIRECTION('',(0.104528463267664,-0.994521895368272,-6.92998990261914E-15));
#127220=DIRECTION('center_axis',(1.4081690688991E-16,6.98296267768627E-15,
-1.));
#127221=DIRECTION('ref_axis',(-1.,-3.28626015289046E-14,-1.4081690689014E-16));
#127222=DIRECTION('',(-1.04744440165294E-14,1.,6.98296267768627E-15));
#127223=DIRECTION('center_axis',(-1.4081690688991E-16,-6.98296267768627E-15,
1.));
#127224=DIRECTION('ref_axis',(-1.,8.32577322149061E-31,-1.39145123902276E-16));
#127225=DIRECTION('center_axis',(0.994633197962181,0.103464010407842,-7.8645720159475E-6));
#127226=DIRECTION('ref_axis',(7.97390952459248E-6,-6.43152286440645E-7,
0.999999999968002));
#127227=DIRECTION('center_axis',(-0.999999427244995,-0.0010702559647401,
-7.86457206393885E-6));
#127228=DIRECTION('ref_axis',(-0.000911792658579952,0.848044334090882,0.529924500330471));
#127229=DIRECTION('center_axis',(-1.4081690688991E-16,-6.98296267768627E-15,
1.));
#127230=DIRECTION('ref_axis',(-1.,8.07722881720021E-31,-1.42096112075504E-16));
#127231=DIRECTION('center_axis',(0.994628478131827,0.103509373458162,9.77058553911475E-6));
#127232=DIRECTION('ref_axis',(0.0905383273445441,-0.869943071289534,-0.484769908303914));
#127233=DIRECTION('center_axis',(-0.999999475000345,-0.00102464802306551,
9.77051628317655E-6));
#127234=DIRECTION('ref_axis',(0.000891471298448989,-0.874648786634207,-0.484756336026909));
#127235=DIRECTION('center_axis',(-1.4081690688991E-16,-6.98296267768627E-15,
1.));
#127236=DIRECTION('ref_axis',(-1.,8.24049048117772E-31,-1.37719829560012E-16));
#127237=DIRECTION('center_axis',(-0.994246940479907,-0.10711218892576,-1.81624797563042E-5));
#127238=DIRECTION('ref_axis',(0.0926692157706902,-0.860268013675041,0.50134953983827));
#127239=DIRECTION('center_axis',(0.999996624262643,-0.00259829454877719,
-1.81316452277342E-5));
#127240=DIRECTION('ref_axis',(0.00224363754548584,0.866978573811876,-0.49834036425087));
#127241=DIRECTION('center_axis',(-1.4081690688991E-16,-6.98296267768627E-15,
1.));
#127242=DIRECTION('ref_axis',(-1.,8.26087817385229E-31,-1.38060560438432E-16));
#127243=DIRECTION('center_axis',(-0.994245493086362,-0.107125623150708,
-1.84940598363496E-5));
#127244=DIRECTION('ref_axis',(0.092885154403067,-0.86199199692417,-0.498339387696979));
#127245=DIRECTION('center_axis',(0.999996589057285,-0.00261180600214046,
-1.85257108111962E-5));
#127246=DIRECTION('ref_axis',(0.00226914104442406,0.865242466403795,0.501348506859647));
#127247=DIRECTION('center_axis',(-1.4081690688991E-16,-6.98296267768627E-15,
1.));
#127248=DIRECTION('ref_axis',(-1.,9.83319205199467E-31,-1.40816906889911E-16));
#127249=DIRECTION('center_axis',(-1.4081690688991E-16,-6.98296267768627E-15,
1.));
#127250=DIRECTION('ref_axis',(-1.,8.46073526001725E-31,-1.4081690688991E-16));
#127251=DIRECTION('',(1.04744440165294E-14,-1.,-6.98296267768627E-15));
#127252=DIRECTION('center_axis',(-1.4081690688991E-16,-6.98296267768627E-15,
1.));
#127253=DIRECTION('ref_axis',(-1.,7.97077743482043E-31,-1.4081690688991E-16));
#127254=DIRECTION('center_axis',(-1.4081690688991E-16,-6.98296267768627E-15,
1.));
#127255=DIRECTION('ref_axis',(-1.,7.97077743482043E-31,-1.4081690688991E-16));
#127256=DIRECTION('center_axis',(-1.4081690688991E-16,-6.98296267768627E-15,
1.));
#127257=DIRECTION('ref_axis',(-1.,7.97077743482043E-31,-1.4081690688991E-16));
#127258=DIRECTION('',(0.104528463267644,0.994521895368274,6.95942865237777E-15));
#127259=DIRECTION('center_axis',(1.4081690688991E-16,6.98296267768627E-15,
-1.));
#127260=DIRECTION('ref_axis',(1.,-7.97077743482043E-31,1.4081690688991E-16));
#127261=DIRECTION('',(4.77800117084862E-6,-0.500005191251989,-0.866022406579779));
#127262=DIRECTION('center_axis',(1.4081690688991E-16,6.98296267768627E-15,
-1.));
#127263=DIRECTION('ref_axis',(-1.,1.15463194561016E-14,-1.4081690688983E-16));
#127264=DIRECTION('',(0.0522695260941882,0.497265611060784,0.86602240657978));
#127265=DIRECTION('center_axis',(-1.4081690688991E-16,-6.98296267768627E-15,
1.));
#127266=DIRECTION('ref_axis',(-1.,9.83319205199467E-31,-1.40816906889911E-16));
#127267=DIRECTION('center_axis',(-1.4081690688991E-16,-6.98296267768627E-15,
1.));
#127268=DIRECTION('ref_axis',(-1.,7.98248735348668E-31,-1.4081690688991E-16));
#127269=DIRECTION('',(1.04744440165294E-14,-1.,-6.98296267768627E-15));
#127270=DIRECTION('center_axis',(1.4081690688991E-16,6.98296267768627E-15,
-1.));
#127271=DIRECTION('ref_axis',(-1.,1.06581410364015E-14,-1.40816906889836E-16));
#127272=DIRECTION('',(0.104528463267644,0.994521895368274,6.95942865237777E-15));
#127273=DIRECTION('center_axis',(-1.4081690688991E-16,-6.98296267768627E-15,
1.));
#127274=DIRECTION('ref_axis',(-1.,7.99150043815584E-31,-1.4081690688991E-16));
#127275=DIRECTION('center_axis',(-1.4081690688991E-16,-6.98296267768627E-15,
1.));
#127276=DIRECTION('ref_axis',(1.,-2.1316282072803E-14,1.40816906889762E-16));
#127277=DIRECTION('',(-4.62770264722375E-6,-0.500004991781227,0.866022521746657));
#127278=DIRECTION('center_axis',(-1.4081690688991E-16,-6.98296267768627E-15,
1.));
#127279=DIRECTION('ref_axis',(-1.,7.99858039355471E-31,-1.4081690688991E-16));
#127280=DIRECTION('center_axis',(-1.4081690688991E-16,-6.98296267768627E-15,
1.));
#127281=DIRECTION('ref_axis',(-1.,7.99858039355471E-31,-1.4081690688991E-16));
#127282=DIRECTION('center_axis',(-1.4081690688991E-16,-6.98296267768627E-15,
1.));
#127283=DIRECTION('ref_axis',(-1.,7.99858039355471E-31,-1.4081690688991E-16));
#127284=DIRECTION('',(0.0522601510654249,0.497266395846527,-0.866022521746648));
#127285=DIRECTION('center_axis',(-1.4081690688991E-16,-6.98296267768627E-15,
1.));
#127286=DIRECTION('ref_axis',(-1.,9.83319205199467E-31,-1.40816906889911E-16));
#127287=DIRECTION('',(1.04744440165294E-14,-1.,-6.98296267768627E-15));
#127288=DIRECTION('center_axis',(1.4081690688991E-16,6.98296267768627E-15,
-1.));
#127289=DIRECTION('ref_axis',(-1.,-3.37507799486048E-14,-1.40816906890146E-16));
#127290=DIRECTION('',(0.104528463267644,0.994521895368274,6.95942865237777E-15));
#127291=DIRECTION('center_axis',(-1.4081690688991E-16,-6.98296267768627E-15,
1.));
#127292=DIRECTION('ref_axis',(-1.,8.32577322149061E-31,-1.39145123902276E-16));
#127293=DIRECTION('center_axis',(0.999999427244995,-0.00107025596495094,
-7.86457221374702E-6));
#127294=DIRECTION('ref_axis',(7.86300009144843E-6,-1.47312952164187E-6,
0.999999999968002));
#127295=DIRECTION('center_axis',(-0.994633197962196,0.103464010407696,-7.86457225038893E-6));
#127296=DIRECTION('ref_axis',(0.0877379732621199,0.843493966781832,0.529924500330476));
#127297=DIRECTION('center_axis',(-1.4081690688991E-16,-6.98296267768627E-15,
1.));
#127298=DIRECTION('ref_axis',(-1.,8.07722881720021E-31,-1.42096112075504E-16));
#127299=DIRECTION('center_axis',(0.999999475000305,-0.00102464806169038,
9.77058611739668E-6));
#127300=DIRECTION('ref_axis',(0.000891463458068991,0.874641264346569,0.484769908302008));
#127301=DIRECTION('center_axis',(-0.994628478127865,0.103509373496238,9.77051631878171E-6));
#127302=DIRECTION('ref_axis',(0.0905391058403046,0.869950553189083,0.484756336028366));
#127303=DIRECTION('center_axis',(-1.4081690688991E-16,-6.98296267768627E-15,
1.));
#127304=DIRECTION('ref_axis',(-1.,8.24049048117772E-31,-1.37719829560012E-16));
#127305=DIRECTION('center_axis',(-0.999996624215829,-0.00259831235054269,
-1.81624797931949E-5));
#127306=DIRECTION('ref_axis',(0.00223907064275388,-0.865241946200867,0.501349539839415));
#127307=DIRECTION('center_axis',(0.994246942387262,-0.107112171226359,-1.81316451653157E-5));
#127308=DIRECTION('ref_axis',(0.0928552846707127,0.861994650485525,-0.498340364252243));
#127309=DIRECTION('center_axis',(-1.4081690688991E-16,-6.98296267768627E-15,
1.));
#127310=DIRECTION('ref_axis',(-1.,8.26087817385229E-31,-1.38060560438432E-16));
#127311=DIRECTION('center_axis',(-0.999996589010146,-0.00261182427508556,
-1.84940601202704E-5));
#127312=DIRECTION('ref_axis',(0.00227362102101954,-0.866979057023569,-0.498339387696754));
#127313=DIRECTION('center_axis',(0.99424549504318,-0.107125604983779,-1.85257088094287E-5));
#127314=DIRECTION('ref_axis',(0.0926991758192284,0.860265387812633,0.501348506863256));
#127315=DIRECTION('center_axis',(-1.4081690688991E-16,-6.98296267768627E-15,
1.));
#127316=DIRECTION('ref_axis',(-1.,9.83319205199467E-31,-1.40816906889911E-16));
#127317=DIRECTION('center_axis',(-1.4081690688991E-16,-6.98296267768627E-15,
1.));
#127318=DIRECTION('ref_axis',(-1.,8.46073526001725E-31,-1.4081690688991E-16));
#127319=DIRECTION('',(-0.104528463267644,-0.994521895368274,-6.95942865237777E-15));
#127320=DIRECTION('center_axis',(-1.4081690688991E-16,-6.98296267768627E-15,
1.));
#127321=DIRECTION('ref_axis',(-1.,7.97077743482043E-31,-1.4081690688991E-16));
#127322=DIRECTION('center_axis',(-1.4081690688991E-16,-6.98296267768627E-15,
1.));
#127323=DIRECTION('ref_axis',(-1.,7.97077743482043E-31,-1.4081690688991E-16));
#127324=DIRECTION('center_axis',(-1.4081690688991E-16,-6.98296267768627E-15,
1.));
#127325=DIRECTION('ref_axis',(-1.,7.97077743482043E-31,-1.4081690688991E-16));
#127326=DIRECTION('',(0.207911690817749,0.978147600733808,6.85964567039975E-15));
#127327=DIRECTION('center_axis',(1.4081690688991E-16,6.98296267768627E-15,
-1.));
#127328=DIRECTION('ref_axis',(1.,-7.97077743482043E-31,1.4081690688991E-16));
#127329=DIRECTION('',(-0.0522600224406443,-0.497266609934999,-0.866022406579794));
#127330=DIRECTION('center_axis',(1.4081690688991E-16,6.98296267768627E-15,
-1.));
#127331=DIRECTION('ref_axis',(-1.,-3.37507799486048E-14,-1.40816906890146E-16));
#127332=DIRECTION('',(0.103961598321227,0.48907788477527,0.866022406579786));
#127333=DIRECTION('center_axis',(-1.4081690688991E-16,-6.98296267768627E-15,
1.));
#127334=DIRECTION('ref_axis',(-1.,9.83319205199467E-31,-1.40816906889911E-16));
#127335=DIRECTION('center_axis',(-1.4081690688991E-16,-6.98296267768627E-15,
1.));
#127336=DIRECTION('ref_axis',(-1.,7.98248735348668E-31,-1.4081690688991E-16));
#127337=DIRECTION('',(-0.104528463267644,-0.994521895368274,-6.95942865237777E-15));
#127338=DIRECTION('center_axis',(1.4081690688991E-16,6.98296267768627E-15,
-1.));
#127339=DIRECTION('ref_axis',(-1.,-3.46389583683049E-14,-1.40816906890152E-16));
#127340=DIRECTION('',(0.207911690817749,0.978147600733808,6.85964567039975E-15));
#127341=DIRECTION('center_axis',(-1.4081690688991E-16,-6.98296267768627E-15,
1.));
#127342=DIRECTION('ref_axis',(-1.,7.99150043815584E-31,-1.4081690688991E-16));
#127343=DIRECTION('center_axis',(-1.4081690688991E-16,-6.98296267768627E-15,
1.));
#127344=DIRECTION('ref_axis',(1.,-1.06581410364015E-14,1.40816906889836E-16));
#127345=DIRECTION('',(-0.0522693557686574,-0.497265428393217,0.866022521746658));
#127346=DIRECTION('center_axis',(-1.4081690688991E-16,-6.98296267768627E-15,
1.));
#127347=DIRECTION('ref_axis',(-1.,7.99858039355471E-31,-1.4081690688991E-16));
#127348=DIRECTION('center_axis',(-1.4081690688991E-16,-6.98296267768627E-15,
1.));
#127349=DIRECTION('ref_axis',(-1.,7.99858039355471E-31,-1.4081690688991E-16));
#127350=DIRECTION('center_axis',(-1.4081690688991E-16,-6.98296267768627E-15,
1.));
#127351=DIRECTION('ref_axis',(-1.,7.99858039355471E-31,-1.4081690688991E-16));
#127352=DIRECTION('',(0.103952356682307,0.489079645219225,-0.866022521746653));
#127353=DIRECTION('center_axis',(-1.4081690688991E-16,-6.98296267768627E-15,
1.));
#127354=DIRECTION('ref_axis',(-1.,9.83319205199467E-31,-1.40816906889911E-16));
#127355=DIRECTION('',(-0.104528463267644,-0.994521895368274,-6.95942865237777E-15));
#127356=DIRECTION('center_axis',(1.4081690688991E-16,6.98296267768627E-15,
-1.));
#127357=DIRECTION('ref_axis',(-1.,1.06581410364015E-14,-1.40816906889836E-16));
#127358=DIRECTION('',(0.207911690817749,0.978147600733808,6.85964567039975E-15));
#127359=DIRECTION('center_axis',(-1.4081690688991E-16,-6.98296267768627E-15,
1.));
#127360=DIRECTION('ref_axis',(-1.,8.32577322149061E-31,-1.39145123902276E-16));
#127361=DIRECTION('center_axis',(0.99440945353958,-0.105592796389062,-7.86457201213219E-6));
#127362=DIRECTION('ref_axis',(7.66594158482965E-6,-2.28696690243272E-6,
0.999999999968001));
#127363=DIRECTION('center_axis',(-0.978369559222146,0.206864703431039,-7.86457226808233E-6));
#127364=DIRECTION('ref_axis',(0.17542646358764,0.829702103060259,0.529924500330489));
#127365=DIRECTION('center_axis',(-1.4081690688991E-16,-6.98296267768627E-15,
1.));
#127366=DIRECTION('ref_axis',(-1.,8.07722881720021E-31,-1.42096112075504E-16));
#127367=DIRECTION('center_axis',(0.994414268357392,-0.1055474433218,9.77058458334715E-6));
#127368=DIRECTION('ref_axis',(0.0923114872004053,0.869756704678088,0.484769908305334));
#127369=DIRECTION('center_axis',(-0.978360123509283,0.206909324660436,9.77051334214024E-6));
#127370=DIRECTION('ref_axis',(0.180977717589009,0.855720959435413,0.484756336027916));
#127371=DIRECTION('center_axis',(-1.4081690688991E-16,-6.98296267768627E-15,
1.));
#127372=DIRECTION('ref_axis',(-1.,8.24049048117772E-31,-1.37719829560012E-16));
#127373=DIRECTION('center_axis',(-0.994790135674094,0.101944031878491,-1.81624797398355E-5));
#127374=DIRECTION('ref_axis',(0.0882156062112462,0.860736106898194,-0.501349539844731));
#127375=DIRECTION('center_axis',(0.977604082951528,-0.210452504541392,-1.81316452147401E-5));
#127376=DIRECTION('ref_axis',(0.182449589865955,0.847566533385627,-0.498340364251598));
#127377=DIRECTION('center_axis',(-1.4081690688991E-16,-6.98296267768627E-15,
1.));
#127378=DIRECTION('ref_axis',(-1.,8.26087817385229E-31,-1.38060560438432E-16));
#127379=DIRECTION('center_axis',(-0.994791513041971,0.101930590293766,-1.84940602080538E-5));
#127380=DIRECTION('ref_axis',(0.0883628226287454,0.862467313146972,0.498339387696903));
#127381=DIRECTION('center_axis',(0.977601239325912,-0.210465713419643,-1.85257069575344E-5));
#127382=DIRECTION('ref_axis',(0.182113579025951,0.845863061615953,0.501348506857301));
#127383=DIRECTION('center_axis',(-1.4081690688991E-16,-6.98296267768627E-15,
1.));
#127384=DIRECTION('ref_axis',(-1.,9.83319205199467E-31,-1.40816906889911E-16));
#127385=DIRECTION('center_axis',(-1.4081690688991E-16,-6.98296267768627E-15,
1.));
#127386=DIRECTION('ref_axis',(-1.,8.46073526001725E-31,-1.4081690688991E-16));
#127387=DIRECTION('',(-0.207911690817749,-0.978147600733808,-6.85964567039975E-15));
#127388=DIRECTION('center_axis',(-1.4081690688991E-16,-6.98296267768627E-15,
1.));
#127389=DIRECTION('ref_axis',(-1.,7.97077743482043E-31,-1.4081690688991E-16));
#127390=DIRECTION('center_axis',(-1.4081690688991E-16,-6.98296267768627E-15,
1.));
#127391=DIRECTION('ref_axis',(-1.,7.97077743482043E-31,-1.4081690688991E-16));
#127392=DIRECTION('center_axis',(-1.4081690688991E-16,-6.98296267768627E-15,
1.));
#127393=DIRECTION('ref_axis',(-1.,7.97077743482043E-31,-1.4081690688991E-16));
#127394=DIRECTION('',(0.309016994374938,0.951056516295157,6.68470697498369E-15));
#127395=DIRECTION('center_axis',(1.4081690688991E-16,6.98296267768627E-15,
-1.));
#127396=DIRECTION('ref_axis',(1.,-7.97077743482043E-31,1.4081690688991E-16));
#127397=DIRECTION('',(-0.103952251140481,-0.489079871579877,-0.866022406579782));
#127398=DIRECTION('center_axis',(1.4081690688991E-16,6.98296267768627E-15,
-1.));
#127399=DIRECTION('ref_axis',(-1.,-3.46389583683049E-14,-1.40816906890152E-16));
#127400=DIRECTION('',(0.154514645521708,0.475531718838049,0.866022406579779));
#127401=DIRECTION('center_axis',(-1.4081690688991E-16,-6.98296267768627E-15,
1.));
#127402=DIRECTION('ref_axis',(-1.,9.83319205199467E-31,-1.40816906889911E-16));
#127403=DIRECTION('center_axis',(-1.4081690688991E-16,-6.98296267768627E-15,
1.));
#127404=DIRECTION('ref_axis',(-1.,7.98248735348668E-31,-1.4081690688991E-16));
#127405=DIRECTION('',(-0.207911690817749,-0.978147600733808,-6.85964567039975E-15));
#127406=DIRECTION('center_axis',(1.4081690688991E-16,6.98296267768627E-15,
-1.));
#127407=DIRECTION('ref_axis',(-1.,-3.5527136788005E-14,-1.40816906890159E-16));
#127408=DIRECTION('',(0.309016994374938,0.951056516295157,6.6847069749837E-15));
#127409=DIRECTION('center_axis',(-1.4081690688991E-16,-6.98296267768627E-15,
1.));
#127410=DIRECTION('ref_axis',(-1.,7.99150043815584E-31,-1.4081690688991E-16));
#127411=DIRECTION('center_axis',(-1.4081690688991E-16,-6.98296267768627E-15,
1.));
#127412=DIRECTION('ref_axis',(1.,-1.06581410364015E-14,1.40816906889836E-16));
#127413=DIRECTION('',(-0.103961409834804,-0.489077720912242,0.866022521746662));
#127414=DIRECTION('center_axis',(-1.4081690688991E-16,-6.98296267768627E-15,
1.));
#127415=DIRECTION('ref_axis',(-1.,7.99858039355471E-31,-1.4081690688991E-16));
#127416=DIRECTION('center_axis',(-1.4081690688991E-16,-6.98296267768627E-15,
1.));
#127417=DIRECTION('ref_axis',(-1.,7.99858039355471E-31,-1.4081690688991E-16));
#127418=DIRECTION('center_axis',(-1.4081690688991E-16,-6.98296267768627E-15,
1.));
#127419=DIRECTION('ref_axis',(-1.,7.99858039355471E-31,-1.4081690688991E-16));
#127420=DIRECTION('',(0.154505638525955,0.475534435652384,-0.866022521746666));
#127421=DIRECTION('center_axis',(-1.4081690688991E-16,-6.98296267768627E-15,
1.));
#127422=DIRECTION('ref_axis',(-1.,9.83319205199467E-31,-1.40816906889911E-16));
#127423=DIRECTION('',(-0.207911690817749,-0.978147600733808,-6.85964567039975E-15));
#127424=DIRECTION('center_axis',(1.4081690688991E-16,6.98296267768627E-15,
-1.));
#127425=DIRECTION('ref_axis',(-1.,8.01265634860448E-31,-1.4081690688991E-16));
#127426=DIRECTION('',(0.309016994374938,0.951056516295157,6.68470697498369E-15));
#127427=DIRECTION('center_axis',(-1.4081690688991E-16,-6.98296267768627E-15,
1.));
#127428=DIRECTION('ref_axis',(-1.,8.32577322149061E-31,-1.39145123902276E-16));
#127429=DIRECTION('center_axis',(0.977924521767629,-0.208958440039405,-7.86457201251932E-6));
#127430=DIRECTION('ref_axis',(7.38489362573485E-6,-3.07574772033552E-6,
0.999999999968002));
#127431=DIRECTION('center_axis',(-0.951386698854271,0.307998943474359,-7.86457228732381E-6));
#127432=DIRECTION('ref_axis',(0.261192944867743,0.806819849471253,0.529924500330472));
#127433=DIRECTION('center_axis',(-1.4081690688991E-16,-6.98296267768627E-15,
1.));
#127434=DIRECTION('ref_axis',(-1.,8.07722881720021E-31,-1.42096112075504E-16));
#127435=DIRECTION('center_axis',(0.977934050896058,-0.208913838705245,9.77058218570699E-6));
#127436=DIRECTION('ref_axis',(0.182720126971887,0.855342908548084,0.484769908302775));
#127437=DIRECTION('center_axis',(-0.951372650642623,0.308042333963641,9.7705129532813E-6));
#127438=DIRECTION('ref_axis',(0.269433499592017,0.832115907779642,0.484756336026318));
#127439=DIRECTION('center_axis',(-1.4081690688991E-16,-6.98296267768627E-15,
1.));
#127440=DIRECTION('ref_axis',(-1.,8.24049048117772E-31,-1.37719829560012E-16));
#127441=DIRECTION('center_axis',(-0.978684518232678,0.205369455961189,-1.81624796489768E-5));
#127442=DIRECTION('ref_axis',(0.177703774423476,0.846799862691456,-0.501349539843592));
#127443=DIRECTION('center_axis',(0.950250388606183,-0.311487076176592,-1.81316452359128E-5));
#127444=DIRECTION('ref_axis',(0.270044939174893,0.823852299982039,-0.498340364249508));
#127445=DIRECTION('center_axis',(-1.4081690688991E-16,-6.98296267768627E-15,
1.));
#127446=DIRECTION('ref_axis',(-1.,8.26087817385229E-31,-1.38060560438432E-16));
#127447=DIRECTION('center_axis',(-0.978687293083712,0.205356231983462,-1.8494057605138E-5));
#127448=DIRECTION('ref_axis',(0.178031144702766,0.848506196905287,0.498339387695926));
#127449=DIRECTION('center_axis',(0.950246179855776,-0.311499915451519,-1.85257140792284E-5));
#127450=DIRECTION('ref_axis',(0.269532707750228,0.822193282702853,0.501348506860385));
#127451=DIRECTION('center_axis',(-1.4081690688991E-16,-6.98296267768627E-15,
1.));
#127452=DIRECTION('ref_axis',(-1.,9.83319205199467E-31,-1.40816906889911E-16));
#127453=DIRECTION('center_axis',(-1.4081690688991E-16,-6.98296267768627E-15,
1.));
#127454=DIRECTION('ref_axis',(-1.,8.46073526001725E-31,-1.4081690688991E-16));
#127455=DIRECTION('',(-0.309016994374938,-0.951056516295157,-6.68470697498369E-15));
#127456=DIRECTION('center_axis',(-1.4081690688991E-16,-6.98296267768627E-15,
1.));
#127457=DIRECTION('ref_axis',(-1.,7.97077743482043E-31,-1.4081690688991E-16));
#127458=DIRECTION('center_axis',(-1.4081690688991E-16,-6.98296267768627E-15,
1.));
#127459=DIRECTION('ref_axis',(-1.,7.97077743482043E-31,-1.4081690688991E-16));
#127460=DIRECTION('center_axis',(-1.4081690688991E-16,-6.98296267768627E-15,
1.));
#127461=DIRECTION('ref_axis',(-1.,7.97077743482043E-31,-1.4081690688991E-16));
#127462=DIRECTION('',(0.406736643075792,0.913545457642605,6.43652923108485E-15));
#127463=DIRECTION('center_axis',(1.4081690688991E-16,6.98296267768627E-15,
-1.));
#127464=DIRECTION('ref_axis',(1.,-7.97077743482043E-31,1.4081690688991E-16));
#127465=DIRECTION('',(-0.154505557223399,-0.475534671805183,-0.866022406579774));
#127466=DIRECTION('center_axis',(1.4081690688991E-16,6.98296267768627E-15,
-1.));
#127467=DIRECTION('ref_axis',(-1.,-3.5527136788005E-14,-1.40816906890159E-16));
#127468=DIRECTION('',(0.20337479793158,0.456775527877798,0.866022406579788));
#127469=DIRECTION('center_axis',(-1.4081690688991E-16,-6.98296267768627E-15,
1.));
#127470=DIRECTION('ref_axis',(-1.,9.83319205199467E-31,-1.40816906889911E-16));
#127471=DIRECTION('center_axis',(-1.4081690688991E-16,-6.98296267768627E-15,
1.));
#127472=DIRECTION('ref_axis',(-1.,7.98248735348668E-31,-1.4081690688991E-16));
#127473=DIRECTION('',(-0.309016994374938,-0.951056516295157,-6.68470697498369E-15));
#127474=DIRECTION('center_axis',(1.4081690688991E-16,6.98296267768627E-15,
-1.));
#127475=DIRECTION('ref_axis',(-1.,-3.5527136788005E-14,-1.40816906890159E-16));
#127476=DIRECTION('',(0.406736643075792,0.913545457642605,6.43652923108485E-15));
#127477=DIRECTION('center_axis',(-1.4081690688991E-16,-6.98296267768627E-15,
1.));
#127478=DIRECTION('ref_axis',(-1.,7.99150043815584E-31,-1.4081690688991E-16));
#127479=DIRECTION('center_axis',(-1.4081690688991E-16,-6.98296267768627E-15,
1.));
#127480=DIRECTION('ref_axis',(1.,1.95399252334028E-14,1.40816906890047E-16));
#127481=DIRECTION('',(-0.154514440939474,-0.47553157557486,0.866022521746665));
#127482=DIRECTION('center_axis',(-1.4081690688991E-16,-6.98296267768627E-15,
1.));
#127483=DIRECTION('ref_axis',(-1.,7.99858039355471E-31,-1.4081690688991E-16));
#127484=DIRECTION('center_axis',(-1.4081690688991E-16,-6.98296267768627E-15,
1.));
#127485=DIRECTION('ref_axis',(-1.,7.99858039355471E-31,-1.4081690688991E-16));
#127486=DIRECTION('center_axis',(-1.4081690688991E-16,-6.98296267768627E-15,
1.));
#127487=DIRECTION('ref_axis',(-1.,7.99858039355471E-31,-1.4081690688991E-16));
#127488=DIRECTION('',(0.203366124261502,0.456779171296608,-0.866022521746657));
#127489=DIRECTION('center_axis',(-1.4081690688991E-16,-6.98296267768627E-15,
1.));
#127490=DIRECTION('ref_axis',(-1.,9.83319205199467E-31,-1.40816906889911E-16));
#127491=DIRECTION('',(-0.309016994374938,-0.951056516295157,-6.68470697498369E-15));
#127492=DIRECTION('center_axis',(1.4081690688991E-16,6.98296267768627E-15,
-1.));
#127493=DIRECTION('ref_axis',(-1.,8.01265634860448E-31,-1.4081690688991E-16));
#127494=DIRECTION('',(0.406736643075792,0.913545457642605,6.43652923108485E-15));
#127495=DIRECTION('center_axis',(-1.4081690688991E-16,-6.98296267768627E-15,
1.));
#127496=DIRECTION('ref_axis',(-1.,8.32577322149061E-31,-1.39145123902276E-16));
#127497=DIRECTION('center_axis',(0.95072524429133,-0.310034691293313,-7.86457201063926E-6));
#127498=DIRECTION('ref_axis',(7.02293521503659E-6,-3.83083005362747E-6,
0.999999999968002));
#127499=DIRECTION('center_axis',(-0.91398024672327,0.405758682640087,-7.86457225127319E-6));
#127500=DIRECTION('ref_axis',(0.344097741585791,0.775097908773505,0.529924500330469));
#127501=DIRECTION('center_axis',(-1.4081690688991E-16,-6.98296267768627E-15,
1.));
#127502=DIRECTION('ref_axis',(-1.,8.07722881720021E-31,-1.42096112075504E-16));
#127503=DIRECTION('center_axis',(0.950739383326639,-0.309991330356541,9.77058507340801E-6));
#127504=DIRECTION('ref_axis',(0.27112684679534,0.831557796518516,0.484769908302987));
#127505=DIRECTION('center_axis',(-0.913961739928689,0.40580036699227,9.770515844718E-6));
#127506=DIRECTION('ref_axis',(0.354937311790399,0.799394020105167,0.484756336027807));
#127507=DIRECTION('center_axis',(-1.4081690688991E-16,-6.98296267768627E-15,
1.));
#127508=DIRECTION('ref_axis',(-1.,8.24049048117772E-31,-1.37719829560012E-16));
#127509=DIRECTION('center_axis',(-0.95185622840662,0.306544809307952,-1.81624796959471E-5));
#127510=DIRECTION('ref_axis',(0.265244982896756,0.8235859019861,-0.501349539840062));
#127511=DIRECTION('center_axis',(0.912485552150601,-0.409108930222327,-1.81316452377115E-5));
#127512=DIRECTION('ref_axis',(0.354681619619059,0.791111768375658,-0.498340364251122));
#127513=DIRECTION('center_axis',(-1.4081690688991E-16,-6.98296267768627E-15,
1.));
#127514=DIRECTION('ref_axis',(-1.,8.26087817385229E-31,-1.38060560438432E-16));
#127515=DIRECTION('center_axis',(-0.951860370340164,0.306531947819237,-1.84940498087876E-5));
#127516=DIRECTION('ref_axis',(0.265748920300266,0.825248669209326,0.498339387694248));
#127517=DIRECTION('center_axis',(0.912480024383678,-0.409121259234423,-1.85257023388232E-5));
#127518=DIRECTION('ref_axis',(0.3539987797255,0.789515382131315,0.501348506860148));
#127519=DIRECTION('center_axis',(-1.4081690688991E-16,-6.98296267768627E-15,
1.));
#127520=DIRECTION('ref_axis',(-1.,9.83319205199467E-31,-1.40816906889911E-16));
#127521=DIRECTION('center_axis',(-1.4081690688991E-16,-6.98296267768627E-15,
1.));
#127522=DIRECTION('ref_axis',(-1.,8.46073526001725E-31,-1.4081690688991E-16));
#127523=DIRECTION('',(-0.406736643075792,-0.913545457642605,-6.43652923108485E-15));
#127524=DIRECTION('center_axis',(-1.4081690688991E-16,-6.98296267768627E-15,
1.));
#127525=DIRECTION('ref_axis',(-1.,7.97077743482043E-31,-1.4081690688991E-16));
#127526=DIRECTION('center_axis',(-1.4081690688991E-16,-6.98296267768627E-15,
1.));
#127527=DIRECTION('ref_axis',(-1.,7.97077743482043E-31,-1.4081690688991E-16));
#127528=DIRECTION('center_axis',(-1.4081690688991E-16,-6.98296267768627E-15,
1.));
#127529=DIRECTION('ref_axis',(-1.,7.97077743482043E-31,-1.4081690688991E-16));
#127530=DIRECTION('',(0.499999999999992,0.866025403784443,6.1178315259999E-15));
#127531=DIRECTION('center_axis',(1.4081690688991E-16,6.98296267768627E-15,
-1.));
#127532=DIRECTION('ref_axis',(1.,-7.97077743482043E-31,1.4081690688991E-16));
#127533=DIRECTION('',(-0.203366068089011,-0.456779414654115,-0.866022406579795));
#127534=DIRECTION('center_axis',(1.4081690688991E-16,6.98296267768627E-15,
-1.));
#127535=DIRECTION('ref_axis',(-1.,1.24344978758018E-14,-1.40816906889824E-16));
#127536=DIRECTION('',(0.250006733496394,0.433014808647735,0.866022406579777));
#127537=DIRECTION('center_axis',(-1.4081690688991E-16,-6.98296267768627E-15,
1.));
#127538=DIRECTION('ref_axis',(-1.,9.83319205199467E-31,-1.40816906889911E-16));
#127539=DIRECTION('center_axis',(-1.4081690688991E-16,-6.98296267768627E-15,
1.));
#127540=DIRECTION('ref_axis',(-1.,7.98248735348668E-31,-1.4081690688991E-16));
#127541=DIRECTION('',(-0.406736643075792,-0.913545457642605,-6.43652923108485E-15));
#127542=DIRECTION('center_axis',(1.4081690688991E-16,6.98296267768627E-15,
-1.));
#127543=DIRECTION('ref_axis',(-1.,1.15463194561016E-14,-1.4081690688983E-16));
#127544=DIRECTION('',(0.499999999999992,0.866025403784443,6.1178315259999E-15));
#127545=DIRECTION('center_axis',(-1.4081690688991E-16,-6.98296267768627E-15,
1.));
#127546=DIRECTION('ref_axis',(-1.,7.99150043815584E-31,-1.4081690688991E-16));
#127547=DIRECTION('center_axis',(-1.4081690688991E-16,-6.98296267768627E-15,
1.));
#127548=DIRECTION('ref_axis',(1.,-1.95399252334028E-14,1.40816906889774E-16));
#127549=DIRECTION('',(-0.203374579494986,-0.456775406784097,0.866022521746669));
#127550=DIRECTION('center_axis',(-1.4081690688991E-16,-6.98296267768627E-15,
1.));
#127551=DIRECTION('ref_axis',(-1.,7.99858039355471E-31,-1.4081690688991E-16));
#127552=DIRECTION('center_axis',(-1.4081690688991E-16,-6.98296267768627E-15,
1.));
#127553=DIRECTION('ref_axis',(-1.,7.99858039355471E-31,-1.4081690688991E-16));
#127554=DIRECTION('center_axis',(-1.4081690688991E-16,-6.98296267768627E-15,
1.));
#127555=DIRECTION('ref_axis',(-1.,7.99858039355471E-31,-1.4081690688991E-16));
#127556=DIRECTION('',(0.249998488182543,0.433019338752906,-0.866022521746657));
#127557=DIRECTION('center_axis',(-1.4081690688991E-16,-6.98296267768627E-15,
1.));
#127558=DIRECTION('ref_axis',(-1.,9.83319205199467E-31,-1.40816906889911E-16));
#127559=DIRECTION('',(-0.406736643075792,-0.913545457642605,-6.43652923108485E-15));
#127560=DIRECTION('center_axis',(1.4081690688991E-16,6.98296267768627E-15,
-1.));
#127561=DIRECTION('ref_axis',(-1.,8.01265634860448E-31,-1.4081690688991E-16));
#127562=DIRECTION('',(0.499999999999992,0.866025403784443,6.1178315259999E-15));
#127563=DIRECTION('center_axis',(-1.4081690688991E-16,-6.98296267768627E-15,
1.));
#127564=DIRECTION('ref_axis',(-1.,8.32577322149061E-31,-1.39145123902276E-16));
#127565=DIRECTION('center_axis',(0.913109622086517,-0.407714137590502,-7.86457206372106E-6));
#127566=DIRECTION('ref_axis',(6.584032128358E-6,-4.54394098313704E-6,0.999999999968002));
#127567=DIRECTION('center_axis',(-0.866560035746507,0.499072844768338,-7.8645722123473E-6));
#127568=DIRECTION('ref_axis',(0.423232531439936,0.734883833187554,0.529924500330482));
#127569=DIRECTION('center_axis',(-1.4081690688991E-16,-6.98296267768627E-15,
1.));
#127570=DIRECTION('ref_axis',(-1.,8.07722881720021E-31,-1.42096112075504E-16));
#127571=DIRECTION('center_axis',(0.913128216118261,-0.407672492122314,9.77058748990148E-6));
#127572=DIRECTION('ref_axis',(0.356563044148465,0.798661963255786,0.484769908302891));
#127573=DIRECTION('center_axis',(-0.866537273131149,0.499112366285359,9.77050983173774E-6));
#127574=DIRECTION('ref_axis',(0.436552356526714,0.757913804265093,0.484756336023973));
#127575=DIRECTION('center_axis',(-1.4081690688991E-16,-6.98296267768627E-15,
1.));
#127576=DIRECTION('ref_axis',(-1.,8.24049048117772E-31,-1.37719829560012E-16));
#127577=DIRECTION('center_axis',(-0.914599202553454,0.404361593575243,-1.81624798752258E-5));
#127578=DIRECTION('ref_axis',(0.349880111830903,0.791348561790119,-0.501349539840125));
#127579=DIRECTION('center_axis',(0.864723333035747,-0.502248501217069,-1.81316451772243E-5));
#127580=DIRECTION('ref_axis',(0.435432334017907,0.749703650686303,-0.49834036424852));
#127581=DIRECTION('center_axis',(-1.4081690688991E-16,-6.98296267768627E-15,
1.));
#127582=DIRECTION('ref_axis',(-1.,8.26087817385229E-31,-1.38060560438432E-16));
#127583=DIRECTION('center_axis',(-0.914604666190226,0.404349235489615,-1.84940430890388E-5));
#127584=DIRECTION('ref_axis',(0.350555095114317,0.792949544396151,0.498339387698112));
#127585=DIRECTION('center_axis',(0.864716546819225,-0.502260184878149,-1.85257070796717E-5));
#127586=DIRECTION('ref_axis',(0.434586366990895,0.748187385816106,0.501348506860563));
#127587=DIRECTION('center_axis',(-1.4081690688991E-16,-6.98296267768627E-15,
1.));
#127588=DIRECTION('ref_axis',(-1.,9.83319205199467E-31,-1.40816906889911E-16));
#127589=DIRECTION('center_axis',(-1.4081690688991E-16,-6.98296267768627E-15,
1.));
#127590=DIRECTION('ref_axis',(-1.,8.46073526001725E-31,-1.4081690688991E-16));
#127591=DIRECTION('',(-0.499999999999992,-0.866025403784443,-6.1178315259999E-15));
#127592=DIRECTION('center_axis',(-1.4081690688991E-16,-6.98296267768627E-15,
1.));
#127593=DIRECTION('ref_axis',(-1.,7.97077743482043E-31,-1.4081690688991E-16));
#127594=DIRECTION('center_axis',(-1.4081690688991E-16,-6.98296267768627E-15,
1.));
#127595=DIRECTION('ref_axis',(-1.,7.97077743482043E-31,-1.4081690688991E-16));
#127596=DIRECTION('center_axis',(-1.4081690688991E-16,-6.98296267768627E-15,
1.));
#127597=DIRECTION('ref_axis',(-1.,7.97077743482043E-31,-1.4081690688991E-16));
#127598=DIRECTION('',(0.587785252292466,0.809016994374953,5.73210557847754E-15));
#127599=DIRECTION('center_axis',(1.4081690688991E-16,6.98296267768627E-15,
-1.));
#127600=DIRECTION('ref_axis',(1.,-7.97077743482043E-31,1.4081690688991E-16));
#127601=DIRECTION('',(-0.249998457755584,-0.433019586648885,-0.866022406579794));
#127602=DIRECTION('center_axis',(1.4081690688991E-16,6.98296267768627E-15,
-1.));
#127603=DIRECTION('ref_axis',(-1.,-3.10862446895044E-14,-1.40816906890128E-16));
#127604=DIRECTION('',(0.29389954297172,0.404509888559958,0.866022406579775));
#127605=DIRECTION('center_axis',(-1.4081690688991E-16,-6.98296267768627E-15,
1.));
#127606=DIRECTION('ref_axis',(-1.,9.83319205199467E-31,-1.40816906889911E-16));
#127607=DIRECTION('center_axis',(-1.4081690688991E-16,-6.98296267768627E-15,
1.));
#127608=DIRECTION('ref_axis',(-1.,7.98248735348668E-31,-1.4081690688991E-16));
#127609=DIRECTION('',(-0.499999999999992,-0.866025403784443,-6.1178315259999E-15));
#127610=DIRECTION('center_axis',(1.4081690688991E-16,6.98296267768627E-15,
-1.));
#127611=DIRECTION('ref_axis',(-1.,-3.01980662698043E-14,-1.40816906890121E-16));
#127612=DIRECTION('',(0.587785252292466,0.809016994374953,5.73210557847754E-15));
#127613=DIRECTION('center_axis',(-1.4081690688991E-16,-6.98296267768627E-15,
1.));
#127614=DIRECTION('ref_axis',(-1.,7.99150043815584E-31,-1.4081690688991E-16));
#127615=DIRECTION('center_axis',(-1.4081690688991E-16,-6.98296267768627E-15,
1.));
#127616=DIRECTION('ref_axis',(1.,-1.95399252334028E-14,1.40816906889774E-16));
#127617=DIRECTION('',(-0.250006503598662,-0.433014711050211,0.866022521746677));
#127618=DIRECTION('center_axis',(-1.4081690688991E-16,-6.98296267768627E-15,
1.));
#127619=DIRECTION('ref_axis',(-1.,7.99858039355471E-31,-1.4081690688991E-16));
#127620=DIRECTION('center_axis',(-1.4081690688991E-16,-6.98296267768627E-15,
1.));
#127621=DIRECTION('ref_axis',(-1.,7.99858039355471E-31,-1.4081690688991E-16));
#127622=DIRECTION('center_axis',(-1.4081690688991E-16,-6.98296267768627E-15,
1.));
#127623=DIRECTION('ref_axis',(-1.,7.99858039355471E-31,-1.4081690688991E-16));
#127624=DIRECTION('',(0.293891816351498,0.404515255718706,-0.866022521746661));
#127625=DIRECTION('center_axis',(-1.4081690688991E-16,-6.98296267768627E-15,
1.));
#127626=DIRECTION('ref_axis',(-1.,9.83319205199467E-31,-1.40816906889911E-16));
#127627=DIRECTION('',(-0.499999999999992,-0.866025403784443,-6.1178315259999E-15));
#127628=DIRECTION('center_axis',(1.4081690688991E-16,6.98296267768627E-15,
-1.));
#127629=DIRECTION('ref_axis',(-1.,6.21724893790088E-15,-1.40816906889867E-16));
#127630=DIRECTION('',(0.587785252292466,0.809016994374953,5.73210557847754E-15));
#127631=DIRECTION('center_axis',(-1.4081690688991E-16,-6.98296267768627E-15,
1.));
#127632=DIRECTION('ref_axis',(-1.,8.32577322149061E-31,-1.39145123902276E-16));
#127633=DIRECTION('center_axis',(0.865489779781638,-0.500926582476595,-7.86457211857109E-6));
#127634=DIRECTION('ref_axis',(6.07299298702999E-6,-5.20726759105563E-6,
0.999999999968002));
#127635=DIRECTION('center_axis',(-0.809645611678775,0.586919060371574,-7.86457229727694E-6));
#127636=DIRECTION('ref_axis',(0.497730297112449,0.686618216540942,0.529924500330461));
#127637=DIRECTION('center_axis',(-1.4081690688991E-16,-6.98296267768627E-15,
1.));
#127638=DIRECTION('ref_axis',(-1.,8.07722881720021E-31,-1.42096112075504E-16));
#127639=DIRECTION('center_axis',(0.865512625090237,-0.500887108752004,9.77058713545332E-6));
#127640=DIRECTION('ref_axis',(0.438092662173875,0.757015822392123,0.484769908304326));
#127641=DIRECTION('center_axis',(-0.809618842639359,0.586955986039705,9.77052025762384E-6));
#127642=DIRECTION('ref_axis',(0.513384442288844,0.70812972617887,0.484756336026268));
#127643=DIRECTION('center_axis',(-1.4081690688991E-16,-6.98296267768627E-15,
1.));
#127644=DIRECTION('ref_axis',(-1.,8.24049048117772E-31,-1.37719829560012E-16));
#127645=DIRECTION('center_axis',(-0.867321636444838,0.497748107605415,-1.81624797475569E-5));
#127646=DIRECTION('ref_axis',(0.430681881043011,0.75044104115131,-0.501349539839213));
#127647=DIRECTION('center_axis',(0.807487024129225,-0.589885332530122,-1.81316451447921E-5));
#127648=DIRECTION('ref_axis',(0.511412360644474,0.700081622913156,-0.4983403642485));
#127649=DIRECTION('center_axis',(-1.4081690688991E-16,-6.98296267768627E-15,
1.));
#127650=DIRECTION('ref_axis',(-1.,8.26087817385229E-31,-1.38060560438432E-16));
#127651=DIRECTION('center_axis',(-0.867328361918079,0.49773638833269,-1.8494060228585E-5));
#127652=DIRECTION('ref_axis',(0.431520514947816,0.751962698439911,0.498339387700931));
#127653=DIRECTION('center_axis',(0.807479053808643,-0.589896242840296,-1.85256939485199E-5));
#127654=DIRECTION('ref_axis',(0.510412535076595,0.69866209193385,0.501348506860547));
#127655=DIRECTION('center_axis',(-1.4081690688991E-16,-6.98296267768627E-15,
1.));
#127656=DIRECTION('ref_axis',(-1.,9.83319205199467E-31,-1.40816906889911E-16));
#127657=DIRECTION('center_axis',(-1.4081690688991E-16,-6.98296267768627E-15,
1.));
#127658=DIRECTION('ref_axis',(-1.,8.46073526001725E-31,-1.4081690688991E-16));
#127659=DIRECTION('',(-0.587785252292466,-0.809016994374953,-5.73210557847754E-15));
#127660=DIRECTION('center_axis',(-1.4081690688991E-16,-6.98296267768627E-15,
1.));
#127661=DIRECTION('ref_axis',(-1.,7.97077743482043E-31,-1.4081690688991E-16));
#127662=DIRECTION('center_axis',(-1.4081690688991E-16,-6.98296267768627E-15,
1.));
#127663=DIRECTION('ref_axis',(-1.,7.97077743482043E-31,-1.4081690688991E-16));
#127664=DIRECTION('center_axis',(-1.4081690688991E-16,-6.98296267768627E-15,
1.));
#127665=DIRECTION('ref_axis',(-1.,7.97077743482043E-31,-1.4081690688991E-16));
#127666=DIRECTION('',(0.669130606358852,0.7431448254774,5.28357748271718E-15));
#127667=DIRECTION('center_axis',(1.4081690688991E-16,6.98296267768627E-15,
-1.));
#127668=DIRECTION('ref_axis',(1.,-7.97077743482043E-31,1.4081690688991E-16));
#127669=DIRECTION('',(-0.293891812003427,-0.40451550543717,-0.866022406579791));
#127670=DIRECTION('center_axis',(1.4081690688991E-16,6.98296267768627E-15,
-1.));
#127671=DIRECTION('ref_axis',(-1.,-1.24344978758018E-14,-1.40816906889997E-16));
#127672=DIRECTION('',(0.334572327551836,0.371573073483924,0.866022406579794));
#127673=DIRECTION('center_axis',(-1.4081690688991E-16,-6.98296267768627E-15,
1.));
#127674=DIRECTION('ref_axis',(-1.,9.83319205199467E-31,-1.40816906889911E-16));
#127675=DIRECTION('center_axis',(-1.4081690688991E-16,-6.98296267768627E-15,
1.));
#127676=DIRECTION('ref_axis',(-1.,7.98248735348668E-31,-1.4081690688991E-16));
#127677=DIRECTION('',(-0.587785252292466,-0.809016994374953,-5.73210557847754E-15));
#127678=DIRECTION('center_axis',(1.4081690688991E-16,6.98296267768627E-15,
-1.));
#127679=DIRECTION('ref_axis',(-1.,-1.86517468137026E-14,-1.40816906890041E-16));
#127680=DIRECTION('',(0.669130606358852,0.7431448254774,5.28357748271718E-15));
#127681=DIRECTION('center_axis',(-1.4081690688991E-16,-6.98296267768627E-15,
1.));
#127682=DIRECTION('ref_axis',(-1.,7.99150043815584E-31,-1.4081690688991E-16));
#127683=DIRECTION('center_axis',(-1.4081690688991E-16,-6.98296267768627E-15,
1.));
#127684=DIRECTION('ref_axis',(1.,-7.99370576998456E-31,1.4081690688991E-16));
#127685=DIRECTION('',(-0.293899304131726,-0.404509815527901,0.866022521746675));
#127686=DIRECTION('center_axis',(-1.4081690688991E-16,-6.98296267768627E-15,
1.));
#127687=DIRECTION('ref_axis',(-1.,7.99858039355471E-31,-1.4081690688991E-16));
#127688=DIRECTION('center_axis',(-1.4081690688991E-16,-6.98296267768627E-15,
1.));
#127689=DIRECTION('ref_axis',(-1.,7.99858039355471E-31,-1.4081690688991E-16));
#127690=DIRECTION('center_axis',(-1.4081690688991E-16,-6.98296267768627E-15,
1.));
#127691=DIRECTION('ref_axis',(-1.,7.99858039355471E-31,-1.4081690688991E-16));
#127692=DIRECTION('',(0.334565204279777,0.371579218892523,-0.866022521746665));
#127693=DIRECTION('center_axis',(-1.4081690688991E-16,-6.98296267768627E-15,
1.));
#127694=DIRECTION('ref_axis',(-1.,9.83319205199467E-31,-1.40816906889911E-16));
#127695=DIRECTION('',(-0.587785252292466,-0.809016994374953,-5.73210557847754E-15));
#127696=DIRECTION('center_axis',(1.4081690688991E-16,6.98296267768627E-15,
-1.));
#127697=DIRECTION('ref_axis',(-1.,-2.48689957516035E-14,-1.40816906890084E-16));
#127698=DIRECTION('',(0.669130606358852,0.7431448254774,5.28357748271718E-15));
#127699=DIRECTION('center_axis',(-1.4081690688991E-16,-6.98296267768627E-15,
1.));
#127700=DIRECTION('ref_axis',(-1.,8.32577322149061E-31,-1.39145123902276E-16));
#127701=DIRECTION('center_axis',(0.808387450334157,-0.588650770899341,-7.86457196308693E-6));
#127702=DIRECTION('ref_axis',(5.49541666557491E-6,-5.81354219714192E-6,
0.999999999968002));
#127703=DIRECTION('center_axis',(-0.743860540860235,0.668334867928696,-7.86457222760781E-6));
#127704=DIRECTION('ref_axis',(0.566774825493132,0.630829867029739,0.529924500330445));
#127705=DIRECTION('center_axis',(-1.4081690688991E-16,-6.98296267768627E-15,
1.));
#127706=DIRECTION('ref_axis',(-1.,8.07722881720021E-31,-1.42096112075504E-16));
#127707=DIRECTION('center_axis',(0.808414296620605,-0.588613901402225,9.77058976039386E-6));
#127708=DIRECTION('ref_axis',(0.514822445316446,0.707075657763804,0.484769908303186));
#127709=DIRECTION('center_axis',(-0.743830058679867,0.668368793188942,9.77051703262605E-6));
#127710=DIRECTION('ref_axis',(0.58459178066967,0.650587230628417,0.484756336025339));
#127711=DIRECTION('center_axis',(-1.4081690688991E-16,-6.98296267768627E-15,
1.));
#127712=DIRECTION('ref_axis',(-1.,8.24049048117772E-31,-1.37719829560012E-16));
#127713=DIRECTION('center_axis',(-0.810541512988669,0.585681189208057,-1.81624797215642E-5));
#127714=DIRECTION('ref_axis',(0.506765009439602,0.701311531424528,-0.501349539840881));
#127715=DIRECTION('center_axis',(0.741403718408774,-0.671059256698607,-1.81316451549613E-5));
#127716=DIRECTION('ref_axis',(0.581789246428761,0.642789354378738,-0.498340364246385));
#127717=DIRECTION('center_axis',(-1.4081690688991E-16,-6.98296267768627E-15,
1.));
#127718=DIRECTION('ref_axis',(-1.,8.26087817385229E-31,-1.38060560438432E-16));
#127719=DIRECTION('center_axis',(-0.810549426627886,0.585670237122544,-1.84940269143515E-5));
#127720=DIRECTION('ref_axis',(0.507758105719755,0.702737191804305,0.498339387697667));
#127721=DIRECTION('center_axis',(0.741394651314913,-0.671069274112917,-1.85257001779312E-5));
#127722=DIRECTION('ref_axis',(0.580646516616626,0.641482109967152,0.501348506862311));
#127723=DIRECTION('center_axis',(-1.4081690688991E-16,-6.98296267768627E-15,
1.));
#127724=DIRECTION('ref_axis',(-1.,9.83319205199467E-31,-1.40816906889911E-16));
#127725=DIRECTION('center_axis',(-1.4081690688991E-16,-6.98296267768627E-15,
1.));
#127726=DIRECTION('ref_axis',(-1.,8.46073526001725E-31,-1.4081690688991E-16));
#127727=DIRECTION('',(-0.669130606358852,-0.7431448254774,-5.28357748271718E-15));
#127728=DIRECTION('center_axis',(-1.4081690688991E-16,-6.98296267768627E-15,
1.));
#127729=DIRECTION('ref_axis',(-1.,7.97077743482043E-31,-1.4081690688991E-16));
#127730=DIRECTION('center_axis',(-1.4081690688991E-16,-6.98296267768627E-15,
1.));
#127731=DIRECTION('ref_axis',(-1.,7.97077743482043E-31,-1.4081690688991E-16));
#127732=DIRECTION('center_axis',(-1.4081690688991E-16,-6.98296267768627E-15,
1.));
#127733=DIRECTION('ref_axis',(-1.,7.97077743482043E-31,-1.4081690688991E-16));
#127734=DIRECTION('',(0.743144825477389,0.669130606358864,4.7771614063965E-15));
#127735=DIRECTION('center_axis',(1.4081690688991E-16,6.98296267768627E-15,
-1.));
#127736=DIRECTION('ref_axis',(1.,-7.97077743482043E-31,1.4081690688991E-16));
#127737=DIRECTION('',(-0.334565226058174,-0.371579467697563,-0.866022406579783));
#127738=DIRECTION('center_axis',(1.4081690688991E-16,6.98296267768627E-15,
-1.));
#127739=DIRECTION('ref_axis',(-1.,-7.105427357601E-15,-1.4081690688996E-16));
#127740=DIRECTION('',(0.371579467697516,0.334565226058181,0.8660224065798));
#127741=DIRECTION('center_axis',(-1.4081690688991E-16,-6.98296267768627E-15,
1.));
#127742=DIRECTION('ref_axis',(-1.,9.83319205199467E-31,-1.40816906889911E-16));
#127743=DIRECTION('center_axis',(-1.4081690688991E-16,-6.98296267768627E-15,
1.));
#127744=DIRECTION('ref_axis',(-1.,7.98248735348668E-31,-1.4081690688991E-16));
#127745=DIRECTION('',(-0.669130606358852,-0.7431448254774,-5.28357748271718E-15));
#127746=DIRECTION('center_axis',(1.4081690688991E-16,6.98296267768627E-15,
-1.));
#127747=DIRECTION('ref_axis',(-1.,-1.24344978758018E-14,-1.40816906889997E-16));
#127748=DIRECTION('',(0.743144825477389,0.669130606358864,4.7771614063965E-15));
#127749=DIRECTION('center_axis',(-1.4081690688991E-16,-6.98296267768627E-15,
1.));
#127750=DIRECTION('ref_axis',(-1.,7.99150043815584E-31,-1.4081690688991E-16));
#127751=DIRECTION('center_axis',(-1.4081690688991E-16,-6.98296267768627E-15,
1.));
#127752=DIRECTION('ref_axis',(1.,-7.99370576998456E-31,1.4081690688991E-16));
#127753=DIRECTION('',(-0.334572082386297,-0.3715730258176,0.866022521746663));
#127754=DIRECTION('center_axis',(-1.4081690688991E-16,-6.98296267768627E-15,
1.));
#127755=DIRECTION('ref_axis',(-1.,7.99858039355471E-31,-1.4081690688991E-16));
#127756=DIRECTION('center_axis',(-1.4081690688991E-16,-6.98296267768627E-15,
1.));
#127757=DIRECTION('ref_axis',(-1.,7.99858039355471E-31,-1.4081690688991E-16));
#127758=DIRECTION('center_axis',(-1.4081690688991E-16,-6.98296267768627E-15,
1.));
#127759=DIRECTION('ref_axis',(-1.,7.99858039355471E-31,-1.4081690688991E-16));
#127760=DIRECTION('',(0.371573025817624,0.334572082386294,-0.866022521746654));
#127761=DIRECTION('center_axis',(-1.4081690688991E-16,-6.98296267768627E-15,
1.));
#127762=DIRECTION('ref_axis',(-1.,9.83319205199467E-31,-1.40816906889911E-16));
#127763=DIRECTION('',(-0.669130606358852,-0.7431448254774,-5.28357748271718E-15));
#127764=DIRECTION('center_axis',(1.4081690688991E-16,6.98296267768627E-15,
-1.));
#127765=DIRECTION('ref_axis',(-1.,3.19744231092045E-14,-1.40816906889687E-16));
#127766=DIRECTION('',(0.743144825477389,0.669130606358864,4.7771614063965E-15));
#127767=DIRECTION('center_axis',(-1.4081690688991E-16,-6.98296267768627E-15,
1.));
#127768=DIRECTION('ref_axis',(-1.,8.32577322149061E-31,-1.39145123902276E-16));
#127769=DIRECTION('center_axis',(0.742428258814862,-0.669925578293053,-7.86457193367171E-6));
#127770=DIRECTION('ref_axis',(4.85763156055902E-6,-6.35612241976888E-6,
0.999999999968002));
#127771=DIRECTION('center_axis',(-0.669925578293245,0.742428258814688,-7.8645722999317E-6));
#127772=DIRECTION('ref_axis',(0.62960965028034,0.568130013485787,0.529924500330479));
#127773=DIRECTION('center_axis',(-1.4081690688991E-16,-6.98296267768627E-15,
1.));
#127774=DIRECTION('ref_axis',(-1.,8.07722881720021E-31,-1.42096112075504E-16));
#127775=DIRECTION('center_axis',(0.742458811944968,-0.669891716973573,9.77059356059858E-6));
#127776=DIRECTION('ref_axis',(0.58591172601474,0.649388624263935,0.484769908301889));
#127777=DIRECTION('center_axis',(-0.669891716941096,0.742458811974272,9.77051458249057E-6));
#127778=DIRECTION('ref_axis',(0.649394209167476,0.585916765234689,0.484756336025292));
#127779=DIRECTION('center_axis',(-1.4081690688991E-16,-6.98296267768627E-15,
1.));
#127780=DIRECTION('ref_axis',(-1.,8.24049048117772E-31,-1.37719829560012E-16));
#127781=DIRECTION('center_axis',(-0.744880927099486,0.667197425140066,-1.81624797614567E-5));
#127782=DIRECTION('ref_axis',(0.577295914344388,0.644498305799741,-0.501349539844748));
#127783=DIRECTION('center_axis',(0.667197438400691,-0.74488091522256,-1.81316453281971E-5));
#127784=DIRECTION('ref_axis',(0.645791927480724,0.578454551164035,-0.498340364247516));
#127785=DIRECTION('center_axis',(-1.4081690688991E-16,-6.98296267768627E-15,
1.));
#127786=DIRECTION('ref_axis',(-1.,8.26087817385229E-31,-1.38060560438432E-16));
#127787=DIRECTION('center_axis',(-0.744889942180744,0.66718736026392,-1.84940550609695E-5));
#127788=DIRECTION('ref_axis',(0.578432592428213,0.645812349435011,0.4983393877008));
#127789=DIRECTION('center_axis',(0.667187373873416,-0.744889929990125,-1.85257023897959E-5));
#127790=DIRECTION('ref_axis',(0.644518813414346,0.577273915766852,0.501348506859419));
#127791=DIRECTION('center_axis',(-1.4081690688991E-16,-6.98296267768627E-15,
1.));
#127792=DIRECTION('ref_axis',(-1.,9.83319205199467E-31,-1.40816906889911E-16));
#127793=DIRECTION('center_axis',(-1.4081690688991E-16,-6.98296267768627E-15,
1.));
#127794=DIRECTION('ref_axis',(-1.,8.46073526001725E-31,-1.4081690688991E-16));
#127795=DIRECTION('',(-0.743144825477389,-0.669130606358864,-4.7771614063965E-15));
#127796=DIRECTION('center_axis',(-1.4081690688991E-16,-6.98296267768627E-15,
1.));
#127797=DIRECTION('ref_axis',(-1.,7.97077743482043E-31,-1.4081690688991E-16));
#127798=DIRECTION('center_axis',(-1.4081690688991E-16,-6.98296267768627E-15,
1.));
#127799=DIRECTION('ref_axis',(-1.,7.97077743482043E-31,-1.4081690688991E-16));
#127800=DIRECTION('center_axis',(-1.4081690688991E-16,-6.98296267768627E-15,
1.));
#127801=DIRECTION('ref_axis',(-1.,7.97077743482043E-31,-1.4081690688991E-16));
#127802=DIRECTION('',(0.809016994374943,0.58778525229248,4.21840575002205E-15));
#127803=DIRECTION('center_axis',(1.4081690688991E-16,6.98296267768627E-15,
-1.));
#127804=DIRECTION('ref_axis',(1.,-7.97077743482043E-31,1.4081690688991E-16));
#127805=DIRECTION('',(-0.371573073483898,-0.334572327551864,-0.866022406579794));
#127806=DIRECTION('center_axis',(1.4081690688991E-16,6.98296267768627E-15,
-1.));
#127807=DIRECTION('ref_axis',(-1.,-1.95399252334028E-14,-1.40816906890047E-16));
#127808=DIRECTION('',(0.404515505437166,0.293891812003465,0.86602240657978));
#127809=DIRECTION('center_axis',(-1.4081690688991E-16,-6.98296267768627E-15,
1.));
#127810=DIRECTION('ref_axis',(-1.,9.83319205199467E-31,-1.40816906889911E-16));
#127811=DIRECTION('center_axis',(-1.4081690688991E-16,-6.98296267768627E-15,
1.));
#127812=DIRECTION('ref_axis',(-1.,7.98248735348668E-31,-1.4081690688991E-16));
#127813=DIRECTION('',(-0.743144825477389,-0.669130606358864,-4.7771614063965E-15));
#127814=DIRECTION('center_axis',(1.4081690688991E-16,6.98296267768627E-15,
-1.));
#127815=DIRECTION('ref_axis',(-1.,-1.33226762955019E-14,-1.40816906890004E-16));
#127816=DIRECTION('',(0.809016994374943,0.58778525229248,4.21840575002205E-15));
#127817=DIRECTION('center_axis',(-1.4081690688991E-16,-6.98296267768627E-15,
1.));
#127818=DIRECTION('ref_axis',(-1.,7.99150043815584E-31,-1.4081690688991E-16));
#127819=DIRECTION('center_axis',(-1.4081690688991E-16,-6.98296267768627E-15,
1.));
#127820=DIRECTION('ref_axis',(1.,-7.99370576998456E-31,1.4081690688991E-16));
#127821=DIRECTION('',(-0.37157921889255,-0.33456520427975,0.866022521746664));
#127822=DIRECTION('center_axis',(-1.4081690688991E-16,-6.98296267768627E-15,
1.));
#127823=DIRECTION('ref_axis',(-1.,7.99858039355471E-31,-1.4081690688991E-16));
#127824=DIRECTION('center_axis',(-1.4081690688991E-16,-6.98296267768627E-15,
1.));
#127825=DIRECTION('ref_axis',(-1.,7.99858039355471E-31,-1.4081690688991E-16));
#127826=DIRECTION('center_axis',(-1.4081690688991E-16,-6.98296267768627E-15,
1.));
#127827=DIRECTION('ref_axis',(-1.,7.99858039355471E-31,-1.4081690688991E-16));
#127828=DIRECTION('',(0.404509815527952,0.293899304131682,-0.866022521746667));
#127829=DIRECTION('center_axis',(-1.4081690688991E-16,-6.98296267768627E-15,
1.));
#127830=DIRECTION('ref_axis',(-1.,9.83319205199467E-31,-1.40816906889911E-16));
#127831=DIRECTION('',(-0.743144825477389,-0.669130606358864,-4.7771614063965E-15));
#127832=DIRECTION('center_axis',(1.4081690688991E-16,6.98296267768627E-15,
-1.));
#127833=DIRECTION('ref_axis',(-1.,-2.57571741713036E-14,-1.4081690689009E-16));
#127834=DIRECTION('',(0.809016994374943,0.58778525229248,4.21840575002205E-15));
#127835=DIRECTION('center_axis',(-1.4081690688991E-16,-6.98296267768627E-15,
1.));
#127836=DIRECTION('ref_axis',(-1.,8.32577322149061E-31,-1.39145123902276E-16));
#127837=DIRECTION('center_axis',(0.668334867928816,-0.743860540860127,-7.86457198807967E-6));
#127838=DIRECTION('ref_axis',(4.16662527142791E-6,-6.82906373300349E-6,
0.999999999968002));
#127839=DIRECTION('center_axis',(-0.58865077089947,0.808387450334064,-7.86457219664369E-6));
#127840=DIRECTION('ref_axis',(0.685546339984931,0.499205608625129,0.529924500330453));
#127841=DIRECTION('center_axis',(-1.4081690688991E-16,-6.98296267768627E-15,
1.));
#127842=DIRECTION('ref_axis',(-1.,8.07722881720021E-31,-1.42096112075504E-16));
#127843=DIRECTION('center_axis',(0.668368793163115,-0.743830058703073,9.77057967136895E-6));
#127844=DIRECTION('ref_axis',(0.650581635231094,0.584586753101467,0.484769908305291));
#127845=DIRECTION('center_axis',(-0.588613901368558,0.808414296645119,9.77051458754715E-6));
#127846=DIRECTION('ref_axis',(0.707081738814029,0.514826873149225,0.484756336027825));
#127847=DIRECTION('center_axis',(-1.4081690688991E-16,-6.98296267768627E-15,
1.));
#127848=DIRECTION('ref_axis',(-1.,8.24049048117772E-31,-1.37719829560012E-16));
#127849=DIRECTION('center_axis',(-0.671059269896464,0.741403706462376,-1.81624794523114E-5));
#127850=DIRECTION('ref_axis',(0.641501844407457,0.580623821869756,-0.501349539841406));
#127851=DIRECTION('center_axis',(0.585681203637541,-0.810541502562901,-1.81316451643526E-5));
#127852=DIRECTION('ref_axis',(0.702719177034256,0.507782078837254,-0.498340364249189));
#127853=DIRECTION('center_axis',(-1.4081690688991E-16,-6.98296267768627E-15,
1.));
#127854=DIRECTION('ref_axis',(-1.,8.26087817385229E-31,-1.38060560438432E-16));
#127855=DIRECTION('center_axis',(-0.671069287648394,0.74139463906414,-1.84940784596614E-5));
#127856=DIRECTION('ref_axis',(0.642769650612951,0.581811851824381,0.49833938769436));
#127857=DIRECTION('center_axis',(0.585670251954522,-0.810549415910174,-1.85257227583356E-5));
#127858=DIRECTION('ref_axis',(0.70132962721531,0.506740987740637,0.501348506862919));
#127859=DIRECTION('center_axis',(-1.4081690688991E-16,-6.98296267768627E-15,
1.));
#127860=DIRECTION('ref_axis',(-1.,9.83319205199467E-31,-1.40816906889911E-16));
#127861=DIRECTION('center_axis',(-1.4081690688991E-16,-6.98296267768627E-15,
1.));
#127862=DIRECTION('ref_axis',(-1.,8.46073526001725E-31,-1.4081690688991E-16));
#127863=DIRECTION('',(-0.809016994374943,-0.58778525229248,-4.21840575002205E-15));
#127864=DIRECTION('center_axis',(-1.4081690688991E-16,-6.98296267768627E-15,
1.));
#127865=DIRECTION('ref_axis',(-1.,7.97077743482043E-31,-1.4081690688991E-16));
#127866=DIRECTION('center_axis',(-1.4081690688991E-16,-6.98296267768627E-15,
1.));
#127867=DIRECTION('ref_axis',(-1.,7.97077743482043E-31,-1.4081690688991E-16));
#127868=DIRECTION('center_axis',(-1.4081690688991E-16,-6.98296267768627E-15,
1.));
#127869=DIRECTION('ref_axis',(-1.,7.97077743482043E-31,-1.4081690688991E-16));
#127870=DIRECTION('',(0.866025403784435,0.500000000000007,3.61343235749219E-15));
#127871=DIRECTION('center_axis',(1.4081690688991E-16,6.98296267768627E-15,
-1.));
#127872=DIRECTION('ref_axis',(1.,-7.97077743482043E-31,1.4081690688991E-16));
#127873=DIRECTION('',(-0.404509888559936,-0.293899542971723,-0.866022406579784));
#127874=DIRECTION('center_axis',(1.4081690688991E-16,6.98296267768627E-15,
-1.));
#127875=DIRECTION('ref_axis',(-1.,3.99680288865056E-14,-1.40816906889631E-16));
#127876=DIRECTION('',(0.433019586648905,0.249998457755594,0.866022406579781));
#127877=DIRECTION('center_axis',(-1.4081690688991E-16,-6.98296267768627E-15,
1.));
#127878=DIRECTION('ref_axis',(-1.,9.83319205199467E-31,-1.40816906889911E-16));
#127879=DIRECTION('center_axis',(-1.4081690688991E-16,-6.98296267768627E-15,
1.));
#127880=DIRECTION('ref_axis',(-1.,7.98248735348668E-31,-1.4081690688991E-16));
#127881=DIRECTION('',(-0.809016994374943,-0.58778525229248,-4.21840575002205E-15));
#127882=DIRECTION('center_axis',(1.4081690688991E-16,6.98296267768627E-15,
-1.));
#127883=DIRECTION('ref_axis',(-1.,3.37507799486048E-14,-1.40816906889675E-16));
#127884=DIRECTION('',(0.866025403784435,0.500000000000007,3.61343235749219E-15));
#127885=DIRECTION('center_axis',(-1.4081690688991E-16,-6.98296267768627E-15,
1.));
#127886=DIRECTION('ref_axis',(-1.,7.99150043815584E-31,-1.4081690688991E-16));
#127887=DIRECTION('center_axis',(-1.4081690688991E-16,-6.98296267768627E-15,
1.));
#127888=DIRECTION('ref_axis',(1.,-7.99370576998456E-31,1.4081690688991E-16));
#127889=DIRECTION('',(-0.404515255718706,-0.293891816351498,0.866022521746661));
#127890=DIRECTION('center_axis',(-1.4081690688991E-16,-6.98296267768627E-15,
1.));
#127891=DIRECTION('ref_axis',(-1.,7.99858039355471E-31,-1.4081690688991E-16));
#127892=DIRECTION('center_axis',(-1.4081690688991E-16,-6.98296267768627E-15,
1.));
#127893=DIRECTION('ref_axis',(-1.,7.99858039355471E-31,-1.4081690688991E-16));
#127894=DIRECTION('center_axis',(-1.4081690688991E-16,-6.98296267768627E-15,
1.));
#127895=DIRECTION('ref_axis',(-1.,7.99858039355471E-31,-1.4081690688991E-16));
#127896=DIRECTION('',(0.433014711050233,0.250006503598672,-0.866022521746663));
#127897=DIRECTION('center_axis',(-1.4081690688991E-16,-6.98296267768627E-15,
1.));
#127898=DIRECTION('ref_axis',(-1.,9.83319205199467E-31,-1.40816906889911E-16));
#127899=DIRECTION('',(-0.809016994374943,-0.58778525229248,-4.21840575002205E-15));
#127900=DIRECTION('center_axis',(1.4081690688991E-16,6.98296267768627E-15,
-1.));
#127901=DIRECTION('ref_axis',(-1.,2.66453525910038E-14,-1.40816906889724E-16));
#127902=DIRECTION('',(0.866025403784435,0.500000000000007,3.61343235749219E-15));
#127903=DIRECTION('center_axis',(-1.4081690688991E-16,-6.98296267768627E-15,
1.));
#127904=DIRECTION('ref_axis',(-1.,8.32577322149061E-31,-1.39145123902276E-16));
#127905=DIRECTION('center_axis',(0.586919060371703,-0.809645611678681,-7.86457199759038E-6));
#127906=DIRECTION('ref_axis',(3.42996853271349E-6,-7.22718433787076E-6,
0.999999999968002));
#127907=DIRECTION('center_axis',(-0.500926582476661,0.865489779781599,-7.86457219974121E-6));
#127908=DIRECTION('ref_axis',(0.733972040528765,0.424811802650939,0.529924500330473));
#127909=DIRECTION('center_axis',(-1.4081690688991E-16,-6.98296267768627E-15,
1.));
#127910=DIRECTION('ref_axis',(-1.,8.07722881720021E-31,-1.42096112075504E-16));
#127911=DIRECTION('center_axis',(0.586955986005525,-0.809618842664138,9.77059659033885E-6));
#127912=DIRECTION('ref_axis',(0.708123635911214,0.513380027141639,0.484769908302828));
#127913=DIRECTION('center_axis',(-0.50088710871783,0.865512625110015,9.77051576765131E-6));
#127914=DIRECTION('ref_axis',(0.757022332964451,0.438096430107843,0.484756336028549));
#127915=DIRECTION('center_axis',(-1.4081690688991E-16,-6.98296267768627E-15,
1.));
#127916=DIRECTION('ref_axis',(-1.,8.24049048117772E-31,-1.37719829560012E-16));
#127917=DIRECTION('center_axis',(-0.589885346904382,0.807487013627849,-1.81624793333984E-5));
#127918=DIRECTION('ref_axis',(0.69867934601742,0.510387901841475,-0.501349539844735));
#127919=DIRECTION('center_axis',(0.497748123045574,-0.867321627584515,-1.81316451742561E-5));
#127920=DIRECTION('ref_axis',(0.751947288231033,0.431546239794873,-0.49834036425008));
#127921=DIRECTION('center_axis',(-1.4081690688991E-16,-6.98296267768627E-15,
1.));
#127922=DIRECTION('ref_axis',(-1.,8.26087817385229E-31,-1.38060560438432E-16));
#127923=DIRECTION('center_axis',(-0.589896257594011,0.80747904303118,-1.84940468888151E-5));
#127924=DIRECTION('ref_axis',(0.700064389995691,0.511436901811145,0.498339387692543));
#127925=DIRECTION('center_axis',(0.497736404187262,-0.867328352818892,-1.85257232350534E-5));
#127926=DIRECTION('ref_axis',(0.750456526860519,0.430656099412363,0.501348506860622));
#127927=DIRECTION('center_axis',(-1.4081690688991E-16,-6.98296267768627E-15,
1.));
#127928=DIRECTION('ref_axis',(-1.,9.83319205199467E-31,-1.40816906889911E-16));
#127929=DIRECTION('center_axis',(-1.4081690688991E-16,-6.98296267768627E-15,
1.));
#127930=DIRECTION('ref_axis',(-1.,8.46073526001725E-31,-1.4081690688991E-16));
#127931=DIRECTION('',(-0.866025403784435,-0.500000000000007,-3.61343235749219E-15));
#127932=DIRECTION('center_axis',(-1.4081690688991E-16,-6.98296267768627E-15,
1.));
#127933=DIRECTION('ref_axis',(-1.,7.97077743482043E-31,-1.4081690688991E-16));
#127934=DIRECTION('center_axis',(-1.4081690688991E-16,-6.98296267768627E-15,
1.));
#127935=DIRECTION('ref_axis',(-1.,7.97077743482043E-31,-1.4081690688991E-16));
#127936=DIRECTION('center_axis',(-1.4081690688991E-16,-6.98296267768627E-15,
1.));
#127937=DIRECTION('ref_axis',(-1.,7.97077743482043E-31,-1.4081690688991E-16));
#127938=DIRECTION('',(0.913545457642598,0.406736643075807,2.96886944389432E-15));
#127939=DIRECTION('center_axis',(1.4081690688991E-16,6.98296267768627E-15,
-1.));
#127940=DIRECTION('ref_axis',(1.,-7.97077743482043E-31,1.4081690688991E-16));
#127941=DIRECTION('',(-0.433014808647732,-0.250006733496379,-0.866022406579783));
#127942=DIRECTION('center_axis',(1.4081690688991E-16,6.98296267768627E-15,
-1.));
#127943=DIRECTION('ref_axis',(-1.,7.10542735760101E-15,-1.40816906889861E-16));
#127944=DIRECTION('',(0.456779414654113,0.203366068089037,0.86602240657979));
#127945=DIRECTION('center_axis',(-1.4081690688991E-16,-6.98296267768627E-15,
1.));
#127946=DIRECTION('ref_axis',(-1.,9.83319205199467E-31,-1.40816906889911E-16));
#127947=DIRECTION('center_axis',(-1.4081690688991E-16,-6.98296267768627E-15,
1.));
#127948=DIRECTION('ref_axis',(-1.,7.98248735348668E-31,-1.4081690688991E-16));
#127949=DIRECTION('',(-0.866025403784435,-0.500000000000007,-3.61343235749219E-15));
#127950=DIRECTION('center_axis',(1.4081690688991E-16,6.98296267768627E-15,
-1.));
#127951=DIRECTION('ref_axis',(-1.,7.10542735760101E-15,-1.40816906889861E-16));
#127952=DIRECTION('',(0.913545457642598,0.406736643075807,2.96886944389432E-15));
#127953=DIRECTION('center_axis',(-1.4081690688991E-16,-6.98296267768627E-15,
1.));
#127954=DIRECTION('ref_axis',(-1.,7.99150043815584E-31,-1.4081690688991E-16));
#127955=DIRECTION('center_axis',(-1.4081690688991E-16,-6.98296267768627E-15,
1.));
#127956=DIRECTION('ref_axis',(1.,-7.99370576998456E-31,1.4081690688991E-16));
#127957=DIRECTION('',(-0.433019338752864,-0.249998488182536,0.86602252174668));
#127958=DIRECTION('center_axis',(-1.4081690688991E-16,-6.98296267768627E-15,
1.));
#127959=DIRECTION('ref_axis',(-1.,7.99858039355471E-31,-1.4081690688991E-16));
#127960=DIRECTION('center_axis',(-1.4081690688991E-16,-6.98296267768627E-15,
1.));
#127961=DIRECTION('ref_axis',(-1.,7.99858039355471E-31,-1.4081690688991E-16));
#127962=DIRECTION('center_axis',(-1.4081690688991E-16,-6.98296267768627E-15,
1.));
#127963=DIRECTION('ref_axis',(-1.,7.99858039355471E-31,-1.4081690688991E-16));
#127964=DIRECTION('',(0.456775406784116,0.203374579494969,-0.866022521746663));
#127965=DIRECTION('center_axis',(-1.4081690688991E-16,-6.98296267768627E-15,
1.));
#127966=DIRECTION('ref_axis',(-1.,9.83319205199467E-31,-1.40816906889911E-16));
#127967=DIRECTION('',(-0.866025403784435,-0.500000000000007,-3.61343235749219E-15));
#127968=DIRECTION('center_axis',(1.4081690688991E-16,6.98296267768627E-15,
-1.));
#127969=DIRECTION('ref_axis',(-1.,8.01265634860448E-31,-1.4081690688991E-16));
#127970=DIRECTION('',(0.913545457642598,0.406736643075807,2.96886944389432E-15));
#127971=DIRECTION('center_axis',(-1.4081690688991E-16,-6.98296267768627E-15,
1.));
#127972=DIRECTION('ref_axis',(-1.,8.32577322149061E-31,-1.39145123902276E-16));
#127973=DIRECTION('center_axis',(0.499072844768409,-0.866560035746466,-7.86457209026023E-6));
#127974=DIRECTION('ref_axis',(2.65573234861323E-6,-7.54612250867244E-6,
0.999999999968002));
#127975=DIRECTION('center_axis',(-0.407714137590658,0.913109622086447,-7.86457230391254E-6));
#127976=DIRECTION('ref_axis',(0.774356189803006,0.345763669669417,0.52992450033048));
#127977=DIRECTION('center_axis',(-1.4081690688991E-16,-6.98296267768627E-15,
1.));
#127978=DIRECTION('ref_axis',(-1.,8.07722881720021E-31,-1.42096112075504E-16));
#127979=DIRECTION('center_axis',(0.499112366251912,-0.866537273150413,9.77057961947491E-6));
#127980=DIRECTION('ref_axis',(0.757907285851233,0.436548602172012,0.484769908302154));
#127981=DIRECTION('center_axis',(-0.407672492090694,0.913128216132379,9.77052487249037E-6));
#127982=DIRECTION('ref_axis',(0.798668832018019,0.356566110900804,0.484756336028782));
#127983=DIRECTION('center_axis',(-1.4081690688991E-16,-6.98296267768627E-15,
1.));
#127984=DIRECTION('ref_axis',(-1.,8.24049048117772E-31,-1.37719829560012E-16));
#127985=DIRECTION('center_axis',(-0.502248516610529,0.864723324094272,-1.81624798592741E-5));
#127986=DIRECTION('ref_axis',(0.74820197050812,0.434560065157779,-0.501349539840054));
#127987=DIRECTION('center_axis',(0.404361609857085,-0.914599195355556,-1.81316452513466E-5));
#127988=DIRECTION('ref_axis',(0.792936907582491,0.350582289842495,-0.498340364251491));
#127989=DIRECTION('center_axis',(-1.4081690688991E-16,-6.98296267768627E-15,
1.));
#127990=DIRECTION('ref_axis',(-1.,8.26087817385229E-31,-1.38060560438432E-16));
#127991=DIRECTION('center_axis',(-0.502260200673814,0.864716537645181,-1.84940675711417E-5));
#127992=DIRECTION('ref_axis',(0.749689077421511,0.435458542074875,0.498339387695682));
#127993=DIRECTION('center_axis',(0.404349252211792,-0.914604658796664,-1.85257124702087E-5));
#127994=DIRECTION('ref_axis',(0.791361267752528,0.349852852737285,0.501348506861938));
#127995=DIRECTION('center_axis',(-1.4081690688991E-16,-6.98296267768627E-15,
1.));
#127996=DIRECTION('ref_axis',(-1.,9.83319205199467E-31,-1.40816906889911E-16));
#127997=DIRECTION('center_axis',(-1.4081690688991E-16,-6.98296267768627E-15,
1.));
#127998=DIRECTION('ref_axis',(-1.,8.46073526001725E-31,-1.4081690688991E-16));
#127999=DIRECTION('',(-0.913545457642598,-0.406736643075807,-2.96886944389432E-15));
#128000=DIRECTION('center_axis',(-1.4081690688991E-16,-6.98296267768627E-15,
1.));
#128001=DIRECTION('ref_axis',(-1.,7.97077743482043E-31,-1.4081690688991E-16));
#128002=DIRECTION('center_axis',(-1.4081690688991E-16,-6.98296267768627E-15,
1.));
#128003=DIRECTION('ref_axis',(-1.,7.97077743482043E-31,-1.4081690688991E-16));
#128004=DIRECTION('center_axis',(-1.4081690688991E-16,-6.98296267768627E-15,
1.));
#128005=DIRECTION('ref_axis',(-1.,7.97077743482043E-31,-1.4081690688991E-16));
#128006=DIRECTION('',(0.951056516295151,0.309016994374955,2.29177897539327E-15));
#128007=DIRECTION('center_axis',(1.4081690688991E-16,6.98296267768627E-15,
-1.));
#128008=DIRECTION('ref_axis',(1.,-7.97077743482043E-31,1.4081690688991E-16));
#128009=DIRECTION('',(-0.456775527877824,-0.20337479793158,-0.866022406579775));
#128010=DIRECTION('center_axis',(1.4081690688991E-16,6.98296267768627E-15,
-1.));
#128011=DIRECTION('ref_axis',(-1.,-2.1316282072803E-14,-1.40816906890059E-16));
#128012=DIRECTION('',(0.475534671805166,0.154505557223409,0.866022406579782));
#128013=DIRECTION('center_axis',(-1.4081690688991E-16,-6.98296267768627E-15,
1.));
#128014=DIRECTION('ref_axis',(-1.,9.83319205199467E-31,-1.40816906889911E-16));
#128015=DIRECTION('center_axis',(-1.4081690688991E-16,-6.98296267768627E-15,
1.));
#128016=DIRECTION('ref_axis',(-1.,7.98248735348668E-31,-1.4081690688991E-16));
#128017=DIRECTION('',(-0.913545457642598,-0.406736643075807,-2.96886944389432E-15));
#128018=DIRECTION('center_axis',(1.4081690688991E-16,6.98296267768627E-15,
-1.));
#128019=DIRECTION('ref_axis',(-1.,-1.77635683940025E-14,-1.40816906890035E-16));
#128020=DIRECTION('',(0.951056516295151,0.309016994374955,2.29177897539327E-15));
#128021=DIRECTION('center_axis',(-1.4081690688991E-16,-6.98296267768627E-15,
1.));
#128022=DIRECTION('ref_axis',(-1.,7.99150043815584E-31,-1.4081690688991E-16));
#128023=DIRECTION('center_axis',(-1.4081690688991E-16,-6.98296267768627E-15,
1.));
#128024=DIRECTION('ref_axis',(1.,-7.99370576998456E-31,1.4081690688991E-16));
#128025=DIRECTION('',(-0.456779171296625,-0.203366124261497,0.866022521746649));
#128026=DIRECTION('center_axis',(-1.4081690688991E-16,-6.98296267768627E-15,
1.));
#128027=DIRECTION('ref_axis',(-1.,7.99858039355471E-31,-1.4081690688991E-16));
#128028=DIRECTION('center_axis',(-1.4081690688991E-16,-6.98296267768627E-15,
1.));
#128029=DIRECTION('ref_axis',(-1.,7.99858039355471E-31,-1.4081690688991E-16));
#128030=DIRECTION('center_axis',(-1.4081690688991E-16,-6.98296267768627E-15,
1.));
#128031=DIRECTION('ref_axis',(-1.,7.99858039355471E-31,-1.4081690688991E-16));
#128032=DIRECTION('',(0.47553157557488,0.154514440939479,-0.866022521746653));
#128033=DIRECTION('center_axis',(-1.4081690688991E-16,-6.98296267768627E-15,
1.));
#128034=DIRECTION('ref_axis',(-1.,9.83319205199467E-31,-1.40816906889911E-16));
#128035=DIRECTION('',(-0.913545457642598,-0.406736643075807,-2.96886944389432E-15));
#128036=DIRECTION('center_axis',(1.4081690688991E-16,6.98296267768627E-15,
-1.));
#128037=DIRECTION('ref_axis',(-1.,-2.04281036531029E-14,-1.40816906890053E-16));
#128038=DIRECTION('',(0.951056516295151,0.309016994374955,2.29177897539327E-15));
#128039=DIRECTION('center_axis',(-1.4081690688991E-16,-6.98296267768627E-15,
1.));
#128040=DIRECTION('ref_axis',(-1.,8.32577322149061E-31,-1.39145123902276E-16));
#128041=DIRECTION('center_axis',(0.405758682640235,-0.913980246723204,-7.86457197116076E-6));
#128042=DIRECTION('ref_axis',(1.85239938593913E-6,-7.78238354702661E-6,
0.999999999968002));
#128043=DIRECTION('center_axis',(-0.310034691293484,0.950725244291274,-7.86457229993127E-6));
#128044=DIRECTION('ref_axis',(0.806256330617376,0.262927277567205,0.529924500330475));
#128045=DIRECTION('center_axis',(-1.4081690688991E-16,-6.98296267768627E-15,
1.));
#128046=DIRECTION('ref_axis',(-1.,8.07722881720021E-31,-1.42096112075504E-16));
#128047=DIRECTION('center_axis',(0.405800366954514,-0.913961739945452,9.77059051480661E-6));
#128048=DIRECTION('ref_axis',(0.799387144964324,0.354934259362841,0.484769908303247));
#128049=DIRECTION('center_axis',(-0.309991330319405,0.950739383338748,9.77051447639857E-6));
#128050=DIRECTION('ref_axis',(0.83156494821626,0.27112917876665,0.484756336028124));
#128051=DIRECTION('center_axis',(-1.4081690688991E-16,-6.98296267768627E-15,
1.));
#128052=DIRECTION('ref_axis',(-1.,8.24049048117772E-31,-1.37719829560012E-16));
#128053=DIRECTION('center_axis',(-0.40910894646611,0.912485544867158,-1.81624798772874E-5));
#128054=DIRECTION('ref_axis',(0.789527137635887,0.353971097460744,-0.501349539841137));
#128055=DIRECTION('center_axis',(0.306544826252958,-0.951856222950077,-1.81316451055346E-5));
#128056=DIRECTION('ref_axis',(0.825238944242033,0.26577728695875,-0.498340364252326));
#128057=DIRECTION('center_axis',(-1.4081690688991E-16,-6.98296267768627E-15,
1.));
#128058=DIRECTION('ref_axis',(-1.,8.26087817385229E-31,-1.38060560438432E-16));
#128059=DIRECTION('center_axis',(-0.409121275907456,0.912480016908768,-1.8494053348855E-5));
#128060=DIRECTION('ref_axis',(0.791100014434309,0.354709207427339,0.498339387695077));
#128061=DIRECTION('center_axis',(0.306531965211348,-0.951860364738688,-1.85256986116291E-5));
#128062=DIRECTION('ref_axis',(0.823595688991342,0.265216544996153,0.501348506864417));
#128063=DIRECTION('center_axis',(-1.4081690688991E-16,-6.98296267768627E-15,
1.));
#128064=DIRECTION('ref_axis',(-1.,9.83319205199467E-31,-1.40816906889911E-16));
#128065=DIRECTION('center_axis',(-1.4081690688991E-16,-6.98296267768627E-15,
1.));
#128066=DIRECTION('ref_axis',(-1.,8.46073526001725E-31,-1.4081690688991E-16));
#128067=DIRECTION('',(-0.951056516295151,-0.309016994374955,-2.29177897539327E-15));
#128068=DIRECTION('center_axis',(-1.4081690688991E-16,-6.98296267768627E-15,
1.));
#128069=DIRECTION('ref_axis',(-1.,7.97077743482043E-31,-1.4081690688991E-16));
#128070=DIRECTION('center_axis',(-1.4081690688991E-16,-6.98296267768627E-15,
1.));
#128071=DIRECTION('ref_axis',(-1.,7.97077743482043E-31,-1.4081690688991E-16));
#128072=DIRECTION('center_axis',(-1.4081690688991E-16,-6.98296267768627E-15,
1.));
#128073=DIRECTION('ref_axis',(-1.,7.97077743482043E-31,-1.4081690688991E-16));
#128074=DIRECTION('',(0.978147600733804,0.207911690817766,1.58957929685223E-15));
#128075=DIRECTION('center_axis',(1.4081690688991E-16,6.98296267768627E-15,
-1.));
#128076=DIRECTION('ref_axis',(1.,-7.97077743482043E-31,1.4081690688991E-16));
#128077=DIRECTION('',(-0.475531718838049,-0.154514645521701,-0.86602240657978));
#128078=DIRECTION('center_axis',(1.4081690688991E-16,6.98296267768627E-15,
-1.));
#128079=DIRECTION('ref_axis',(-1.,4.08562073062058E-14,-1.40816906889625E-16));
#128080=DIRECTION('',(0.489079871579876,0.10395225114048,0.866022406579783));
#128081=DIRECTION('center_axis',(-1.4081690688991E-16,-6.98296267768627E-15,
1.));
#128082=DIRECTION('ref_axis',(-1.,9.83319205199467E-31,-1.40816906889911E-16));
#128083=DIRECTION('center_axis',(-1.4081690688991E-16,-6.98296267768627E-15,
1.));
#128084=DIRECTION('ref_axis',(-1.,7.98248735348668E-31,-1.4081690688991E-16));
#128085=DIRECTION('',(-0.951056516295151,-0.309016994374955,-2.29177897539327E-15));
#128086=DIRECTION('center_axis',(1.4081690688991E-16,6.98296267768627E-15,
-1.));
#128087=DIRECTION('ref_axis',(-1.,3.28626015289046E-14,-1.40816906889681E-16));
#128088=DIRECTION('',(0.978147600733804,0.207911690817766,1.58957929685223E-15));
#128089=DIRECTION('center_axis',(-1.4081690688991E-16,-6.98296267768627E-15,
1.));
#128090=DIRECTION('ref_axis',(-1.,7.99150043815584E-31,-1.4081690688991E-16));
#128091=DIRECTION('center_axis',(-1.4081690688991E-16,-6.98296267768627E-15,
1.));
#128092=DIRECTION('ref_axis',(1.,-7.99370576998456E-31,1.4081690688991E-16));
#128093=DIRECTION('',(-0.475534435652379,-0.154505638525953,0.866022521746669));
#128094=DIRECTION('center_axis',(-1.4081690688991E-16,-6.98296267768627E-15,
1.));
#128095=DIRECTION('ref_axis',(-1.,7.99858039355471E-31,-1.4081690688991E-16));
#128096=DIRECTION('center_axis',(-1.4081690688991E-16,-6.98296267768627E-15,
1.));
#128097=DIRECTION('ref_axis',(-1.,7.99858039355471E-31,-1.4081690688991E-16));
#128098=DIRECTION('center_axis',(-1.4081690688991E-16,-6.98296267768627E-15,
1.));
#128099=DIRECTION('ref_axis',(-1.,7.99858039355471E-31,-1.4081690688991E-16));
#128100=DIRECTION('',(0.489077720912261,0.103961409834809,-0.86602252174665));
#128101=DIRECTION('center_axis',(-1.4081690688991E-16,-6.98296267768627E-15,
1.));
#128102=DIRECTION('ref_axis',(-1.,9.83319205199467E-31,-1.40816906889911E-16));
#128103=DIRECTION('',(-0.951056516295151,-0.309016994374955,-2.29177897539327E-15));
#128104=DIRECTION('center_axis',(1.4081690688991E-16,6.98296267768627E-15,
-1.));
#128105=DIRECTION('ref_axis',(-1.,2.48689957516035E-14,-1.40816906889737E-16));
#128106=DIRECTION('',(0.978147600733804,0.207911690817766,1.58957929685223E-15));
#128107=DIRECTION('center_axis',(-1.4081690688991E-16,-6.98296267768627E-15,
1.));
#128108=DIRECTION('ref_axis',(-1.,8.32577322149061E-31,-1.39145123902276E-16));
#128109=DIRECTION('center_axis',(0.307998943474541,-0.951386698854212,-7.86457199095568E-6));
#128110=DIRECTION('ref_axis',(1.02877118498534E-6,-7.93337931236483E-6,
0.999999999968002));
#128111=DIRECTION('center_axis',(-0.208958440039579,0.977924521767592,-7.86457230358117E-6));
#128112=DIRECTION('ref_axis',(0.829322958353489,0.177210199190901,0.529924500330508));
#128113=DIRECTION('center_axis',(-1.4081690688991E-16,-6.98296267768627E-15,
1.));
#128114=DIRECTION('ref_axis',(-1.,8.07722881720021E-31,-1.42096112075504E-16));
#128115=DIRECTION('center_axis',(0.308042333923395,-0.951372650655653,9.77058934107909E-6));
#128116=DIRECTION('ref_axis',(0.832108751234113,0.269431182533241,0.484769908305316));
#128117=DIRECTION('center_axis',(-0.20891383867053,0.977934050903475,9.77051809992799E-6));
#128118=DIRECTION('ref_axis',(0.85535026482736,0.182721698612803,0.484756336024417));
#128119=DIRECTION('center_axis',(-1.4081690688991E-16,-6.98296267768627E-15,
1.));
#128120=DIRECTION('ref_axis',(-1.,8.24049048117772E-31,-1.37719829560012E-16));
#128121=DIRECTION('center_axis',(-0.311487093092621,0.950250383060608,-1.81624796851363E-5));
#128122=DIRECTION('ref_axis',(0.822202080224231,0.269503948346828,-0.50134953984263));
#128123=DIRECTION('center_axis',(0.205369473383632,-0.978684514577284,-1.81316452252925E-5));
#128124=DIRECTION('ref_axis',(0.84849949033903,0.17806037250233,-0.498340364247908));
#128125=DIRECTION('center_axis',(-1.4081690688991E-16,-6.98296267768627E-15,
1.));
#128126=DIRECTION('ref_axis',(-1.,8.26087817385229E-31,-1.38060560438432E-16));
#128127=DIRECTION('center_axis',(-0.311499932813636,0.950246174164921,-1.84940668588953E-5));
#128128=DIRECTION('ref_axis',(0.823843494140552,0.270073604475409,0.498339387694719));
#128129=DIRECTION('center_axis',(0.20535624986749,-0.97868728933054,-1.8525709393338E-5));
#128130=DIRECTION('ref_axis',(0.846806623518089,0.177674469289194,0.501348506857951));
#128131=DIRECTION('center_axis',(-1.4081690688991E-16,-6.98296267768627E-15,
1.));
#128132=DIRECTION('ref_axis',(-1.,9.83319205199467E-31,-1.40816906889911E-16));
#128133=DIRECTION('center_axis',(-1.4081690688991E-16,-6.98296267768627E-15,
1.));
#128134=DIRECTION('ref_axis',(-1.,8.46073526001725E-31,-1.4081690688991E-16));
#128135=DIRECTION('',(-0.978147600733804,-0.207911690817766,-1.58957929685223E-15));
#128136=DIRECTION('center_axis',(-1.4081690688991E-16,-6.98296267768627E-15,
1.));
#128137=DIRECTION('ref_axis',(-1.,7.97077743482043E-31,-1.4081690688991E-16));
#128138=DIRECTION('center_axis',(-1.4081690688991E-16,-6.98296267768627E-15,
1.));
#128139=DIRECTION('ref_axis',(-1.,7.97077743482043E-31,-1.4081690688991E-16));
#128140=DIRECTION('center_axis',(-1.4081690688991E-16,-6.98296267768627E-15,
1.));
#128141=DIRECTION('ref_axis',(-1.,7.97077743482043E-31,-1.4081690688991E-16));
#128142=DIRECTION('',(0.994521895368273,0.104528463267661,8.69963854894025E-16));
#128143=DIRECTION('center_axis',(1.4081690688991E-16,6.98296267768627E-15,
-1.));
#128144=DIRECTION('ref_axis',(1.,-7.97077743482043E-31,1.4081690688991E-16));
#128145=DIRECTION('',(-0.48907788477529,-0.103961598321232,-0.866022406579774));
#128146=DIRECTION('center_axis',(1.4081690688991E-16,6.98296267768627E-15,
-1.));
#128147=DIRECTION('ref_axis',(-1.,-1.68753899743024E-14,-1.40816906890028E-16));
#128148=DIRECTION('',(0.497266609935039,0.0522600224406394,0.866022406579771));
#128149=DIRECTION('center_axis',(-1.4081690688991E-16,-6.98296267768627E-15,
1.));
#128150=DIRECTION('ref_axis',(-1.,9.83319205199467E-31,-1.40816906889911E-16));
#128151=DIRECTION('center_axis',(-1.4081690688991E-16,-6.98296267768627E-15,
1.));
#128152=DIRECTION('ref_axis',(-1.,7.98248735348668E-31,-1.4081690688991E-16));
#128153=DIRECTION('',(-0.978147600733804,-0.207911690817766,-1.58957929685223E-15));
#128154=DIRECTION('center_axis',(1.4081690688991E-16,6.98296267768627E-15,
-1.));
#128155=DIRECTION('ref_axis',(-1.,-2.22044604925031E-14,-1.40816906890066E-16));
#128156=DIRECTION('',(0.994521895368273,0.104528463267661,8.69963854894025E-16));
#128157=DIRECTION('center_axis',(-1.4081690688991E-16,-6.98296267768627E-15,
1.));
#128158=DIRECTION('ref_axis',(-1.,7.99150043815584E-31,-1.4081690688991E-16));
#128159=DIRECTION('center_axis',(-1.4081690688991E-16,-6.98296267768627E-15,
1.));
#128160=DIRECTION('ref_axis',(1.,-7.99370576998456E-31,1.4081690688991E-16));
#128161=DIRECTION('',(-0.489079645219224,-0.103952356682314,0.866022521746652));
#128162=DIRECTION('center_axis',(-1.4081690688991E-16,-6.98296267768627E-15,
1.));
#128163=DIRECTION('ref_axis',(-1.,7.99858039355471E-31,-1.4081690688991E-16));
#128164=DIRECTION('center_axis',(-1.4081690688991E-16,-6.98296267768627E-15,
1.));
#128165=DIRECTION('ref_axis',(-1.,7.99858039355471E-31,-1.4081690688991E-16));
#128166=DIRECTION('center_axis',(-1.4081690688991E-16,-6.98296267768627E-15,
1.));
#128167=DIRECTION('ref_axis',(-1.,7.99858039355471E-31,-1.4081690688991E-16));
#128168=DIRECTION('',(0.497265428393237,0.0522693557686703,-0.866022521746645));
#128169=DIRECTION('center_axis',(-1.4081690688991E-16,-6.98296267768627E-15,
1.));
#128170=DIRECTION('ref_axis',(-1.,9.83319205199467E-31,-1.40816906889911E-16));
#128171=DIRECTION('',(-0.978147600733804,-0.207911690817766,-1.58957929685223E-15));
#128172=DIRECTION('center_axis',(1.4081690688991E-16,6.98296267768627E-15,
-1.));
#128173=DIRECTION('ref_axis',(-1.,-2.39808173319034E-14,-1.40816906890078E-16));
#128174=DIRECTION('',(0.994521895368273,0.104528463267661,8.69963854894025E-16));
#128175=DIRECTION('center_axis',(-1.4081690688991E-16,-6.98296267768627E-15,
1.));
#128176=DIRECTION('ref_axis',(-1.,8.32577322149061E-31,-1.39145123902276E-16));
#128177=DIRECTION('center_axis',(0.206864703431171,-0.978369559222118,-7.86457205940785E-6));
#128178=DIRECTION('ref_axis',(1.93871496019899E-7,-7.99745537400948E-6,
0.999999999968001));
#128179=DIRECTION('center_axis',(-0.105592796389226,0.994409453539563,-7.86457227510478E-6));
#128180=DIRECTION('ref_axis',(0.843303350210945,0.0895515687886275,0.529924500330464));
#128181=DIRECTION('center_axis',(-1.4081690688991E-16,-6.98296267768627E-15,
1.));
#128182=DIRECTION('ref_axis',(-1.,8.07722881720021E-31,-1.42096112075504E-16));
#128183=DIRECTION('center_axis',(0.206909324622084,-0.978360123517393,9.77058419069398E-6));
#128184=DIRECTION('ref_axis',(0.855713599897009,0.180976161286358,0.484769908304296));
#128185=DIRECTION('center_axis',(-0.105547443284138,0.99441426836139,9.77051615051766E-6));
#128186=DIRECTION('ref_axis',(0.869764184940149,0.0923122812911752,0.484756336026892));
#128187=DIRECTION('center_axis',(-1.4081690688991E-16,-6.98296267768627E-15,
1.));
#128188=DIRECTION('ref_axis',(-1.,8.24049048117772E-31,-1.37719829560012E-16));
#128189=DIRECTION('center_axis',(-0.2104525219444,0.977604079204545,-1.81624797895158E-5));
#128190=DIRECTION('ref_axis',(0.845868804765923,0.182084057577827,-0.501349539842078));
#128191=DIRECTION('center_axis',(0.101944049587683,-0.994790133859855,-1.81316451673808E-5));
#128192=DIRECTION('ref_axis',(0.862463698457448,0.0883925913424541,-0.498340364248037));
#128193=DIRECTION('center_axis',(-1.4081690688991E-16,-6.98296267768627E-15,
1.));
#128194=DIRECTION('ref_axis',(-1.,8.26087817385229E-31,-1.38060560438432E-16));
#128195=DIRECTION('center_axis',(-0.210465731280713,0.977601235481239,-1.84940611137989E-5));
#128196=DIRECTION('ref_axis',(0.847560772121457,0.182479018595617,0.49833938770005));
#128197=DIRECTION('center_axis',(0.101930608471618,-0.994791511178802,-1.8525711081838E-5));
#128198=DIRECTION('ref_axis',(0.860739767467695,0.0881857549147744,0.50134850685902));
#128199=DIRECTION('center_axis',(-1.4081690688991E-16,-6.98296267768627E-15,
1.));
#128200=DIRECTION('ref_axis',(-1.,9.83319205199467E-31,-1.40816906889911E-16));
#128201=DIRECTION('center_axis',(-1.4081690688991E-16,-6.98296267768627E-15,
1.));
#128202=DIRECTION('ref_axis',(-1.,8.46073526001725E-31,-1.4081690688991E-16));
#128203=DIRECTION('',(-0.994521895368273,-0.104528463267661,-8.69963854894025E-16));
#128204=DIRECTION('center_axis',(-1.4081690688991E-16,-6.98296267768627E-15,
1.));
#128205=DIRECTION('ref_axis',(-1.,7.97077743482043E-31,-1.4081690688991E-16));
#128206=DIRECTION('center_axis',(-1.4081690688991E-16,-6.98296267768627E-15,
1.));
#128207=DIRECTION('ref_axis',(-1.,7.97077743482043E-31,-1.4081690688991E-16));
#128208=DIRECTION('center_axis',(-1.4081690688991E-16,-6.98296267768627E-15,
1.));
#128209=DIRECTION('ref_axis',(-1.,7.97077743482043E-31,-1.4081690688991E-16));
#128210=DIRECTION('',(1.,-9.83319205199467E-31,1.40816906889911E-16));
#128211=DIRECTION('center_axis',(1.4081690688991E-16,6.98296267768627E-15,
-1.));
#128212=DIRECTION('ref_axis',(1.,-7.97077743482043E-31,1.4081690688991E-16));
#128213=DIRECTION('',(-0.497265611060784,-0.0522695260941848,-0.86602240657978));
#128214=DIRECTION('center_axis',(1.4081690688991E-16,6.98296267768627E-15,
-1.));
#128215=DIRECTION('ref_axis',(-1.,-5.32907051820075E-15,-1.40816906889948E-16));
#128216=DIRECTION('',(0.500005191251989,-4.77800117170159E-6,0.866022406579779));
#128217=DIRECTION('center_axis',(-1.4081690688991E-16,-6.98296267768627E-15,
1.));
#128218=DIRECTION('ref_axis',(-1.,9.83319205199467E-31,-1.40816906889911E-16));
#128219=DIRECTION('center_axis',(-1.4081690688991E-16,-6.98296267768627E-15,
1.));
#128220=DIRECTION('ref_axis',(-1.,7.98248735348668E-31,-1.4081690688991E-16));
#128221=DIRECTION('',(-0.994521895368273,-0.104528463267661,-8.69963854894025E-16));
#128222=DIRECTION('center_axis',(1.4081690688991E-16,6.98296267768627E-15,
-1.));
#128223=DIRECTION('ref_axis',(-1.,-1.24344978758018E-14,-1.40816906889997E-16));
#128224=DIRECTION('',(1.,-9.83319205199467E-31,1.40816906889911E-16));
#128225=DIRECTION('center_axis',(-1.4081690688991E-16,-6.98296267768627E-15,
1.));
#128226=DIRECTION('ref_axis',(-1.,7.99150043815584E-31,-1.4081690688991E-16));
#128227=DIRECTION('center_axis',(-1.4081690688991E-16,-6.98296267768627E-15,
1.));
#128228=DIRECTION('ref_axis',(1.,-7.99370576998456E-31,1.4081690688991E-16));
#128229=DIRECTION('',(-0.497266395846526,-0.0522601510654453,0.866022521746648));
#128230=DIRECTION('center_axis',(-1.4081690688991E-16,-6.98296267768627E-15,
1.));
#128231=DIRECTION('ref_axis',(-1.,7.99858039355471E-31,-1.4081690688991E-16));
#128232=DIRECTION('center_axis',(-1.4081690688991E-16,-6.98296267768627E-15,
1.));
#128233=DIRECTION('ref_axis',(-1.,7.99858039355471E-31,-1.4081690688991E-16));
#128234=DIRECTION('center_axis',(-1.4081690688991E-16,-6.98296267768627E-15,
1.));
#128235=DIRECTION('ref_axis',(-1.,7.99858039355471E-31,-1.4081690688991E-16));
#128236=DIRECTION('',(0.500004991781227,4.62770265895213E-6,-0.866022521746658));
#128237=DIRECTION('center_axis',(-1.4081690688991E-16,-6.98296267768627E-15,
1.));
#128238=DIRECTION('ref_axis',(-1.,9.83319205199467E-31,-1.40816906889911E-16));
#128239=DIRECTION('',(-0.994521895368273,-0.104528463267661,-8.69963854894025E-16));
#128240=DIRECTION('center_axis',(1.4081690688991E-16,6.98296267768627E-15,
-1.));
#128241=DIRECTION('ref_axis',(-1.,-1.86517468137026E-14,-1.40816906890041E-16));
#128242=DIRECTION('',(1.,-9.83319205199467E-31,1.40816906889911E-16));
#128243=DIRECTION('center_axis',(-1.4081690688991E-16,-6.98296267768627E-15,
1.));
#128244=DIRECTION('ref_axis',(-1.,8.32577322149061E-31,-1.39145123902276E-16));
#128245=DIRECTION('center_axis',(0.10346401040783,-0.994633197962182,-7.86457203728972E-6));
#128246=DIRECTION('ref_axis',(-6.43152314414477E-7,-7.97390954906981E-6,
0.999999999968001));
#128247=DIRECTION('center_axis',(-0.00107025596492904,0.999999427244995,
-7.86457228206508E-6));
#128248=DIRECTION('ref_axis',(0.848044334090877,0.000911792658855751,0.529924500330479));
#128249=DIRECTION('center_axis',(-1.4081690688991E-16,-6.98296267768627E-15,
1.));
#128250=DIRECTION('ref_axis',(-1.,8.07722881720021E-31,-1.42096112075504E-16));
#128251=DIRECTION('center_axis',(0.10350937345709,-0.994628478131939,9.77058738226894E-6));
#128252=DIRECTION('ref_axis',(0.869943071288686,0.0905383273444065,0.484769908305461));
#128253=DIRECTION('center_axis',(-0.00102464802306466,0.999999475000345,
9.7705163072413E-6));
#128254=DIRECTION('ref_axis',(0.874648786633691,0.000891471298436039,0.484756336027841));
#128255=DIRECTION('center_axis',(-1.4081690688991E-16,-6.98296267768627E-15,
1.));
#128256=DIRECTION('ref_axis',(-1.,8.24049048117772E-31,-1.37719829560012E-16));
#128257=DIRECTION('center_axis',(-0.107112188925754,0.994246940479908,-1.81624798062462E-5));
#128258=DIRECTION('ref_axis',(0.86026801367229,0.0926692157703631,-0.501349539843051));
#128259=DIRECTION('center_axis',(-0.00259829454878754,-0.999996624262643,
-1.81316452336422E-5));
#128260=DIRECTION('ref_axis',(0.866978573810612,-0.00224363754548855,-0.49834036425307));
#128261=DIRECTION('center_axis',(-1.4081690688991E-16,-6.98296267768627E-15,
1.));
#128262=DIRECTION('ref_axis',(-1.,8.26087817385229E-31,-1.38060560438432E-16));
#128263=DIRECTION('center_axis',(-0.107125623149976,0.99424549308644,-1.84940610889373E-5));
#128264=DIRECTION('ref_axis',(0.861991996925822,0.0928851544032302,0.498339387694092));
#128265=DIRECTION('center_axis',(-0.00261180600211858,-0.999996589057285,
-1.85257108738633E-5));
#128266=DIRECTION('ref_axis',(0.865242466403372,-0.00226914104443546,0.501348506860378));
#128267=DIRECTION('center_axis',(-1.4081690688991E-16,-6.98296267768627E-15,
1.));
#128268=DIRECTION('ref_axis',(-1.,9.83319205199467E-31,-1.40816906889911E-16));
#128269=DIRECTION('center_axis',(-1.4081690688991E-16,-6.98296267768627E-15,
1.));
#128270=DIRECTION('ref_axis',(-1.,8.46073526001725E-31,-1.4081690688991E-16));
#128271=DIRECTION('',(-1.,9.83319205199467E-31,-1.40816906889911E-16));
#128272=DIRECTION('center_axis',(-1.4081690688991E-16,-6.98296267768627E-15,
1.));
#128273=DIRECTION('ref_axis',(-1.,7.97077743482043E-31,-1.4081690688991E-16));
#128274=DIRECTION('center_axis',(-1.4081690688991E-16,-6.98296267768627E-15,
1.));
#128275=DIRECTION('ref_axis',(-1.,7.97077743482043E-31,-1.4081690688991E-16));
#128276=DIRECTION('center_axis',(-1.4081690688991E-16,-6.98296267768627E-15,
1.));
#128277=DIRECTION('ref_axis',(-1.,7.97077743482043E-31,-1.4081690688991E-16));
#128278=DIRECTION('',(0.994521895368274,-0.104528463267647,-5.89872860613828E-16));
#128279=DIRECTION('center_axis',(1.4081690688991E-16,6.98296267768627E-15,
-1.));
#128280=DIRECTION('ref_axis',(1.,-7.97077743482043E-31,1.4081690688991E-16));
#128281=DIRECTION('',(-0.500005191251989,-4.77800115933347E-6,-0.866022406579779));
#128282=DIRECTION('center_axis',(1.4081690688991E-16,6.98296267768627E-15,
-1.));
#128283=DIRECTION('ref_axis',(-1.,7.97577417048809E-31,-1.40816906889911E-16));
#128284=DIRECTION('',(0.497265611060783,-0.0522695260942018,0.86602240657978));
#128285=DIRECTION('center_axis',(-1.4081690688991E-16,-6.98296267768627E-15,
1.));
#128286=DIRECTION('ref_axis',(-1.,9.83319205199467E-31,-1.40816906889911E-16));
#128287=DIRECTION('center_axis',(-1.4081690688991E-16,-6.98296267768627E-15,
1.));
#128288=DIRECTION('ref_axis',(-1.,7.98248735348668E-31,-1.4081690688991E-16));
#128289=DIRECTION('',(-1.,9.83319205199467E-31,-1.40816906889911E-16));
#128290=DIRECTION('center_axis',(1.4081690688991E-16,6.98296267768627E-15,
-1.));
#128291=DIRECTION('ref_axis',(-1.,7.98707387273907E-31,-1.4081690688991E-16));
#128292=DIRECTION('',(0.994521895368274,-0.104528463267647,-5.89872860613828E-16));
#128293=DIRECTION('center_axis',(-1.4081690688991E-16,-6.98296267768627E-15,
1.));
#128294=DIRECTION('ref_axis',(-1.,7.99150043815584E-31,-1.4081690688991E-16));
#128295=DIRECTION('center_axis',(-1.4081690688991E-16,-6.98296267768627E-15,
1.));
#128296=DIRECTION('ref_axis',(1.,-7.99370576998456E-31,1.4081690688991E-16));
#128297=DIRECTION('',(-0.500004991781227,4.62770264658402E-6,0.866022521746657));
#128298=DIRECTION('center_axis',(-1.4081690688991E-16,-6.98296267768627E-15,
1.));
#128299=DIRECTION('ref_axis',(-1.,7.99858039355471E-31,-1.4081690688991E-16));
#128300=DIRECTION('center_axis',(-1.4081690688991E-16,-6.98296267768627E-15,
1.));
#128301=DIRECTION('ref_axis',(-1.,7.99858039355471E-31,-1.4081690688991E-16));
#128302=DIRECTION('center_axis',(-1.4081690688991E-16,-6.98296267768627E-15,
1.));
#128303=DIRECTION('ref_axis',(-1.,7.99858039355471E-31,-1.4081690688991E-16));
#128304=DIRECTION('',(0.497266395846507,-0.0522601510654256,-0.86602252174666));
#128305=DIRECTION('center_axis',(-1.4081690688991E-16,-6.98296267768627E-15,
1.));
#128306=DIRECTION('ref_axis',(-1.,9.83319205199467E-31,-1.40816906889911E-16));
#128307=DIRECTION('',(-1.,9.83319205199467E-31,-1.40816906889911E-16));
#128308=DIRECTION('center_axis',(1.4081690688991E-16,6.98296267768627E-15,
-1.));
#128309=DIRECTION('ref_axis',(-1.,8.01265634860448E-31,-1.4081690688991E-16));
#128310=DIRECTION('',(0.994521895368274,-0.104528463267647,-5.89872860613828E-16));
#128311=DIRECTION('center_axis',(-1.4081690688991E-16,-6.98296267768627E-15,
1.));
#128312=DIRECTION('ref_axis',(-1.,8.32577322149061E-31,-1.39145123902276E-16));
#128313=DIRECTION('center_axis',(-0.00107025596477632,-0.999999427244995,
-7.86457202049714E-6));
#128314=DIRECTION('ref_axis',(-1.47312953562887E-6,-7.86299989814554E-6,
0.999999999968002));
#128315=DIRECTION('center_axis',(0.103464010407677,0.994633197962198,-7.86457228356451E-6));
#128316=DIRECTION('ref_axis',(0.84349396678185,-0.0877379732620883,0.529924500330452));
#128317=DIRECTION('center_axis',(-1.4081690688991E-16,-6.98296267768627E-15,
1.));
#128318=DIRECTION('ref_axis',(-1.,8.07722881720021E-31,-1.42096112075504E-16));
#128319=DIRECTION('center_axis',(-0.00102464806165045,-0.999999475000305,
9.77058601886064E-6));
#128320=DIRECTION('ref_axis',(0.874641264344646,-0.000891463458079829,0.484769908305479));
#128321=DIRECTION('center_axis',(0.103509373496843,0.994628478127802,9.77051526104263E-6));
#128322=DIRECTION('ref_axis',(0.869950553189323,-0.0905391058403489,0.484756336027927));
#128323=DIRECTION('center_axis',(-1.4081690688991E-16,-6.98296267768627E-15,
1.));
#128324=DIRECTION('ref_axis',(-1.,8.24049048117772E-31,-1.37719829560012E-16));
#128325=DIRECTION('center_axis',(-0.00259831235056312,0.999996624215829,
-1.81624797722911E-5));
#128326=DIRECTION('ref_axis',(0.865241946199094,0.00223907064277737,-0.501349539842474));
#128327=DIRECTION('center_axis',(-0.107112171226389,-0.994246942387258,
-1.81316452158989E-5));
#128328=DIRECTION('ref_axis',(0.861994650487816,-0.0928552846709603,-0.498340364248234));
#128329=DIRECTION('center_axis',(-1.4081690688991E-16,-6.98296267768627E-15,
1.));
#128330=DIRECTION('ref_axis',(-1.,8.26087817385229E-31,-1.38060560438432E-16));
#128331=DIRECTION('center_axis',(-0.0026118242750409,0.999996589010146,
-1.84940601491707E-5));
#128332=DIRECTION('ref_axis',(0.866979057020819,0.00227362102098813,0.498339387701539));
#128333=DIRECTION('center_axis',(-0.107125604983594,-0.9942454950432,-1.85257091479021E-5));
#128334=DIRECTION('ref_axis',(0.860265387815186,-0.0926991758195122,0.501348506858822));
#128335=DIRECTION('center_axis',(-1.4081690688991E-16,-6.98296267768627E-15,
1.));
#128336=DIRECTION('ref_axis',(-1.,9.83319205199467E-31,-1.40816906889911E-16));
#128337=DIRECTION('center_axis',(-1.4081690688991E-16,-6.98296267768627E-15,
1.));
#128338=DIRECTION('ref_axis',(-1.,8.46073526001725E-31,-1.4081690688991E-16));
#128339=DIRECTION('',(-0.994521895368274,0.104528463267647,5.89872860613828E-16));
#128340=DIRECTION('center_axis',(-1.4081690688991E-16,-6.98296267768627E-15,
1.));
#128341=DIRECTION('ref_axis',(-1.,7.97077743482043E-31,-1.4081690688991E-16));
#128342=DIRECTION('center_axis',(-1.4081690688991E-16,-6.98296267768627E-15,
1.));
#128343=DIRECTION('ref_axis',(-1.,7.97077743482043E-31,-1.4081690688991E-16));
#128344=DIRECTION('center_axis',(-1.4081690688991E-16,-6.98296267768627E-15,
1.));
#128345=DIRECTION('ref_axis',(-1.,7.97077743482043E-31,-1.4081690688991E-16));
#128346=DIRECTION('',(0.978147600733807,-0.207911690817753,-1.3140998576179E-15));
#128347=DIRECTION('center_axis',(1.4081690688991E-16,6.98296267768627E-15,
-1.));
#128348=DIRECTION('ref_axis',(1.,-7.97077743482043E-31,1.4081690688991E-16));
#128349=DIRECTION('',(-0.49726660993504,0.0522600224406429,-0.86602240657977));
#128350=DIRECTION('center_axis',(1.4081690688991E-16,6.98296267768627E-15,
-1.));
#128351=DIRECTION('ref_axis',(-1.,7.97577417048809E-31,-1.40816906889911E-16));
#128352=DIRECTION('',(0.489077884775249,-0.103961598321242,0.866022406579796));
#128353=DIRECTION('center_axis',(-1.4081690688991E-16,-6.98296267768627E-15,
1.));
#128354=DIRECTION('ref_axis',(-1.,9.83319205199467E-31,-1.40816906889911E-16));
#128355=DIRECTION('center_axis',(-1.4081690688991E-16,-6.98296267768627E-15,
1.));
#128356=DIRECTION('ref_axis',(-1.,7.98248735348668E-31,-1.4081690688991E-16));
#128357=DIRECTION('',(-0.994521895368274,0.104528463267647,5.89872860613828E-16));
#128358=DIRECTION('center_axis',(1.4081690688991E-16,6.98296267768627E-15,
-1.));
#128359=DIRECTION('ref_axis',(-1.,7.98707387273907E-31,-1.4081690688991E-16));
#128360=DIRECTION('',(0.978147600733807,-0.207911690817753,-1.3140998576179E-15));
#128361=DIRECTION('center_axis',(-1.4081690688991E-16,-6.98296267768627E-15,
1.));
#128362=DIRECTION('ref_axis',(-1.,7.99150043815584E-31,-1.4081690688991E-16));
#128363=DIRECTION('center_axis',(-1.4081690688991E-16,-6.98296267768627E-15,
1.));
#128364=DIRECTION('ref_axis',(1.,-7.99370576998456E-31,1.4081690688991E-16));
#128365=DIRECTION('',(-0.497265428393217,0.0522693557686506,0.866022521746658));
#128366=DIRECTION('center_axis',(-1.4081690688991E-16,-6.98296267768627E-15,
1.));
#128367=DIRECTION('ref_axis',(-1.,7.99858039355471E-31,-1.4081690688991E-16));
#128368=DIRECTION('center_axis',(-1.4081690688991E-16,-6.98296267768627E-15,
1.));
#128369=DIRECTION('ref_axis',(-1.,7.99858039355471E-31,-1.4081690688991E-16));
#128370=DIRECTION('center_axis',(-1.4081690688991E-16,-6.98296267768627E-15,
1.));
#128371=DIRECTION('ref_axis',(-1.,7.99858039355471E-31,-1.4081690688991E-16));
#128372=DIRECTION('',(0.489079645219225,-0.1039523566823,-0.866022521746653));
#128373=DIRECTION('center_axis',(-1.4081690688991E-16,-6.98296267768627E-15,
1.));
#128374=DIRECTION('ref_axis',(-1.,9.83319205199467E-31,-1.40816906889911E-16));
#128375=DIRECTION('',(-0.994521895368274,0.104528463267647,5.89872860613828E-16));
#128376=DIRECTION('center_axis',(1.4081690688991E-16,6.98296267768627E-15,
-1.));
#128377=DIRECTION('ref_axis',(-1.,8.01265634860448E-31,-1.4081690688991E-16));
#128378=DIRECTION('',(0.978147600733807,-0.207911690817753,-1.3140998576179E-15));
#128379=DIRECTION('center_axis',(-1.4081690688991E-16,-6.98296267768627E-15,
1.));
#128380=DIRECTION('ref_axis',(-1.,8.32577322149061E-31,-1.39145123902276E-16));
#128381=DIRECTION('center_axis',(-0.105592796389069,-0.99440945353958,-7.86457202324616E-6));
#128382=DIRECTION('ref_axis',(-2.28696686047185E-6,-7.66594159881603E-6,
0.999999999968002));
#128383=DIRECTION('center_axis',(0.206864703431021,0.97836955922215,-7.8645722885402E-6));
#128384=DIRECTION('ref_axis',(0.829702103060282,-0.17542646358762,0.529924500330458));
#128385=DIRECTION('center_axis',(-1.4081690688991E-16,-6.98296267768627E-15,
1.));
#128386=DIRECTION('ref_axis',(-1.,8.07722881720021E-31,-1.42096112075504E-16));
#128387=DIRECTION('center_axis',(-0.105547443321967,-0.994414268357374,
9.77058488673039E-6));
#128388=DIRECTION('ref_axis',(0.869756704678642,-0.0923114872004638,0.48476990830433));
#128389=DIRECTION('center_axis',(0.206909324658795,0.97836012350963,9.77051638199737E-6));
#128390=DIRECTION('ref_axis',(0.855720959435164,-0.180977717588963,0.484756336028372));
#128391=DIRECTION('center_axis',(-1.4081690688991E-16,-6.98296267768627E-15,
1.));
#128392=DIRECTION('ref_axis',(-1.,8.24049048117772E-31,-1.37719829560012E-16));
#128393=DIRECTION('center_axis',(0.101944031878469,0.994790135674096,-1.81624797646096E-5));
#128394=DIRECTION('ref_axis',(0.860736106897086,-0.0882156062111255,-0.501349539846655));
#128395=DIRECTION('center_axis',(-0.210452504541414,-0.977604082951524,
-1.81316452978814E-5));
#128396=DIRECTION('ref_axis',(0.847566533387204,-0.182449589866272,-0.4983403642488));
#128397=DIRECTION('center_axis',(-1.4081690688991E-16,-6.98296267768627E-15,
1.));
#128398=DIRECTION('ref_axis',(-1.,8.26087817385229E-31,-1.38060560438432E-16));
#128399=DIRECTION('center_axis',(0.101930590295467,0.994791513041797,-1.84940631498201E-5));
#128400=DIRECTION('ref_axis',(0.862467313147321,-0.088362822628798,0.498339387696289));
#128401=DIRECTION('center_axis',(-0.210465713418178,-0.977601239326227,
-1.85257095408342E-5));
#128402=DIRECTION('ref_axis',(0.845863061613335,-0.182113579025386,0.501348506861923));
#128403=DIRECTION('center_axis',(-1.4081690688991E-16,-6.98296267768627E-15,
1.));
#128404=DIRECTION('ref_axis',(-1.,9.83319205199467E-31,-1.40816906889911E-16));
#128405=DIRECTION('center_axis',(-1.4081690688991E-16,-6.98296267768627E-15,
1.));
#128406=DIRECTION('ref_axis',(-1.,8.46073526001725E-31,-1.4081690688991E-16));
#128407=DIRECTION('',(-0.978147600733807,0.207911690817753,1.3140998576179E-15));
#128408=DIRECTION('center_axis',(-1.4081690688991E-16,-6.98296267768627E-15,
1.));
#128409=DIRECTION('ref_axis',(-1.,7.97077743482043E-31,-1.4081690688991E-16));
#128410=DIRECTION('center_axis',(-1.4081690688991E-16,-6.98296267768627E-15,
1.));
#128411=DIRECTION('ref_axis',(-1.,7.97077743482043E-31,-1.4081690688991E-16));
#128412=DIRECTION('center_axis',(-1.4081690688991E-16,-6.98296267768627E-15,
1.));
#128413=DIRECTION('ref_axis',(-1.,7.97077743482043E-31,-1.4081690688991E-16));
#128414=DIRECTION('',(0.951056516295155,-0.309016994374942,-2.02392930158883E-15));
#128415=DIRECTION('center_axis',(1.4081690688991E-16,6.98296267768627E-15,
-1.));
#128416=DIRECTION('ref_axis',(1.,-7.97077743482043E-31,1.4081690688991E-16));
#128417=DIRECTION('',(-0.489079871579896,0.103952251140493,-0.86602240657977));
#128418=DIRECTION('center_axis',(1.4081690688991E-16,6.98296267768627E-15,
-1.));
#128419=DIRECTION('ref_axis',(-1.,7.97577417048809E-31,-1.40816906889911E-16));
#128420=DIRECTION('',(0.475531718838027,-0.15451464552171,0.86602240657979));
#128421=DIRECTION('center_axis',(-1.4081690688991E-16,-6.98296267768627E-15,
1.));
#128422=DIRECTION('ref_axis',(-1.,9.83319205199467E-31,-1.40816906889911E-16));
#128423=DIRECTION('center_axis',(-1.4081690688991E-16,-6.98296267768627E-15,
1.));
#128424=DIRECTION('ref_axis',(-1.,7.98248735348668E-31,-1.4081690688991E-16));
#128425=DIRECTION('',(-0.978147600733807,0.207911690817753,1.3140998576179E-15));
#128426=DIRECTION('center_axis',(1.4081690688991E-16,6.98296267768627E-15,
-1.));
#128427=DIRECTION('ref_axis',(-1.,7.98707387273907E-31,-1.4081690688991E-16));
#128428=DIRECTION('',(0.951056516295155,-0.309016994374942,-2.02392930158883E-15));
#128429=DIRECTION('center_axis',(-1.4081690688991E-16,-6.98296267768627E-15,
1.));
#128430=DIRECTION('ref_axis',(-1.,7.99150043815584E-31,-1.4081690688991E-16));
#128431=DIRECTION('center_axis',(-1.4081690688991E-16,-6.98296267768627E-15,
1.));
#128432=DIRECTION('ref_axis',(1.,-7.99370576998456E-31,1.4081690688991E-16));
#128433=DIRECTION('',(-0.489077720912262,0.103961409834795,0.866022521746651));
#128434=DIRECTION('center_axis',(-1.4081690688991E-16,-6.98296267768627E-15,
1.));
#128435=DIRECTION('ref_axis',(-1.,7.99858039355471E-31,-1.4081690688991E-16));
#128436=DIRECTION('center_axis',(-1.4081690688991E-16,-6.98296267768627E-15,
1.));
#128437=DIRECTION('ref_axis',(-1.,7.99858039355471E-31,-1.4081690688991E-16));
#128438=DIRECTION('center_axis',(-1.4081690688991E-16,-6.98296267768627E-15,
1.));
#128439=DIRECTION('ref_axis',(-1.,7.99858039355471E-31,-1.4081690688991E-16));
#128440=DIRECTION('',(0.475534435652402,-0.154505638525938,-0.86602252174666));
#128441=DIRECTION('center_axis',(-1.4081690688991E-16,-6.98296267768627E-15,
1.));
#128442=DIRECTION('ref_axis',(-1.,9.83319205199467E-31,-1.40816906889911E-16));
#128443=DIRECTION('',(-0.978147600733807,0.207911690817753,1.3140998576179E-15));
#128444=DIRECTION('center_axis',(1.4081690688991E-16,6.98296267768627E-15,
-1.));
#128445=DIRECTION('ref_axis',(-1.,8.01265634860448E-31,-1.4081690688991E-16));
#128446=DIRECTION('',(0.951056516295155,-0.309016994374942,-2.02392930158883E-15));
#128447=DIRECTION('center_axis',(-1.4081690688991E-16,-6.98296267768627E-15,
1.));
#128448=DIRECTION('ref_axis',(-1.,8.32577322149061E-31,-1.39145123902276E-16));
#128449=DIRECTION('center_axis',(-0.208958440039409,-0.977924521767629,
-7.8645720061062E-6));
#128450=DIRECTION('ref_axis',(-3.07574767837472E-6,-7.38489362573465E-6,
0.999999999968001));
#128451=DIRECTION('center_axis',(0.30799894347438,0.951386698854264,-7.86457224109976E-6));
#128452=DIRECTION('ref_axis',(0.806819849471229,-0.26119294486778,0.529924500330491));
#128453=DIRECTION('center_axis',(-1.4081690688991E-16,-6.98296267768627E-15,
1.));
#128454=DIRECTION('ref_axis',(-1.,8.07722881720021E-31,-1.42096112075504E-16));
#128455=DIRECTION('center_axis',(-0.208913838705841,-0.977934050895931,
9.77058339197564E-6));
#128456=DIRECTION('ref_axis',(0.855342908547101,-0.182720126971624,0.484769908304609));
#128457=DIRECTION('center_axis',(0.308042333962524,0.951372650642984,9.77051511636161E-6));
#128458=DIRECTION('ref_axis',(0.832115907779852,-0.269433499592107,0.484756336025908));
#128459=DIRECTION('center_axis',(-1.4081690688991E-16,-6.98296267768627E-15,
1.));
#128460=DIRECTION('ref_axis',(-1.,8.24049048117772E-31,-1.37719829560012E-16));
#128461=DIRECTION('center_axis',(0.205369455961115,0.978684518232694,-1.81624798107456E-5));
#128462=DIRECTION('ref_axis',(0.846799862691689,-0.177703774423541,-0.501349539843176));
#128463=DIRECTION('center_axis',(-0.311487076176515,-0.950250388606208,
-1.81316450997518E-5));
#128464=DIRECTION('ref_axis',(0.8238522999842,-0.270044939175598,-0.498340364245554));
#128465=DIRECTION('center_axis',(-1.4081690688991E-16,-6.98296267768627E-15,
1.));
#128466=DIRECTION('ref_axis',(-1.,8.26087817385229E-31,-1.38060560438432E-16));
#128467=DIRECTION('center_axis',(0.205356231983588,0.978687293083686,-1.84940578039158E-5));
#128468=DIRECTION('ref_axis',(0.84850619690631,-0.178031144702993,0.498339387694101));
#128469=DIRECTION('center_axis',(-0.311499915462665,-0.950246179852122,
-1.85256937060462E-5));
#128470=DIRECTION('ref_axis',(0.822193282703536,-0.269532707750384,0.50134850685918));
#128471=DIRECTION('center_axis',(-1.4081690688991E-16,-6.98296267768627E-15,
1.));
#128472=DIRECTION('ref_axis',(-1.,9.83319205199467E-31,-1.40816906889911E-16));
#128473=DIRECTION('center_axis',(-1.4081690688991E-16,-6.98296267768627E-15,
1.));
#128474=DIRECTION('ref_axis',(-1.,8.46073526001725E-31,-1.4081690688991E-16));
#128475=DIRECTION('',(-0.951056516295155,0.309016994374942,2.02392930158883E-15));
#128476=DIRECTION('center_axis',(-1.4081690688991E-16,-6.98296267768627E-15,
1.));
#128477=DIRECTION('ref_axis',(-1.,7.97077743482043E-31,-1.4081690688991E-16));
#128478=DIRECTION('center_axis',(-1.4081690688991E-16,-6.98296267768627E-15,
1.));
#128479=DIRECTION('ref_axis',(-1.,7.97077743482043E-31,-1.4081690688991E-16));
#128480=DIRECTION('center_axis',(-1.4081690688991E-16,-6.98296267768627E-15,
1.));
#128481=DIRECTION('ref_axis',(-1.,7.97077743482043E-31,-1.4081690688991E-16));
#128482=DIRECTION('',(0.913545457642603,-0.406736643075795,-2.71158415259712E-15));
#128483=DIRECTION('center_axis',(1.4081690688991E-16,6.98296267768627E-15,
-1.));
#128484=DIRECTION('ref_axis',(1.,-7.97077743482043E-31,1.4081690688991E-16));
#128485=DIRECTION('',(-0.475534671805145,0.154505557223411,-0.866022406579793));
#128486=DIRECTION('center_axis',(1.4081690688991E-16,6.98296267768627E-15,
-1.));
#128487=DIRECTION('ref_axis',(-1.,7.97577417048809E-31,-1.40816906889911E-16));
#128488=DIRECTION('',(0.456775527877802,-0.203374797931582,0.866022406579786));
#128489=DIRECTION('center_axis',(-1.4081690688991E-16,-6.98296267768627E-15,
1.));
#128490=DIRECTION('ref_axis',(-1.,9.83319205199467E-31,-1.40816906889911E-16));
#128491=DIRECTION('center_axis',(-1.4081690688991E-16,-6.98296267768627E-15,
1.));
#128492=DIRECTION('ref_axis',(-1.,7.98248735348668E-31,-1.4081690688991E-16));
#128493=DIRECTION('',(-0.951056516295155,0.309016994374942,2.02392930158883E-15));
#128494=DIRECTION('center_axis',(1.4081690688991E-16,6.98296267768627E-15,
-1.));
#128495=DIRECTION('ref_axis',(-1.,7.98707387273907E-31,-1.4081690688991E-16));
#128496=DIRECTION('',(0.913545457642603,-0.406736643075795,-2.71158415259712E-15));
#128497=DIRECTION('center_axis',(-1.4081690688991E-16,-6.98296267768627E-15,
1.));
#128498=DIRECTION('ref_axis',(-1.,7.99150043815584E-31,-1.4081690688991E-16));
#128499=DIRECTION('center_axis',(-1.4081690688991E-16,-6.98296267768627E-15,
1.));
#128500=DIRECTION('ref_axis',(1.,-7.99370576998456E-31,1.4081690688991E-16));
#128501=DIRECTION('',(-0.47553157557486,0.154514440939468,0.866022521746666));
#128502=DIRECTION('center_axis',(-1.4081690688991E-16,-6.98296267768627E-15,
1.));
#128503=DIRECTION('ref_axis',(-1.,7.99858039355471E-31,-1.4081690688991E-16));
#128504=DIRECTION('center_axis',(-1.4081690688991E-16,-6.98296267768627E-15,
1.));
#128505=DIRECTION('ref_axis',(-1.,7.99858039355471E-31,-1.4081690688991E-16));
#128506=DIRECTION('center_axis',(-1.4081690688991E-16,-6.98296267768627E-15,
1.));
#128507=DIRECTION('ref_axis',(-1.,7.99858039355471E-31,-1.4081690688991E-16));
#128508=DIRECTION('',(0.456779171296619,-0.203366124261481,-0.866022521746656));
#128509=DIRECTION('center_axis',(-1.4081690688991E-16,-6.98296267768627E-15,
1.));
#128510=DIRECTION('ref_axis',(-1.,9.83319205199467E-31,-1.40816906889911E-16));
#128511=DIRECTION('',(-0.951056516295155,0.309016994374942,2.02392930158883E-15));
#128512=DIRECTION('center_axis',(1.4081690688991E-16,6.98296267768627E-15,
-1.));
#128513=DIRECTION('ref_axis',(-1.,8.01265634860448E-31,-1.4081690688991E-16));
#128514=DIRECTION('',(0.913545457642603,-0.406736643075795,-2.71158415259712E-15));
#128515=DIRECTION('center_axis',(-1.4081690688991E-16,-6.98296267768627E-15,
1.));
#128516=DIRECTION('ref_axis',(-1.,8.32577322149061E-31,-1.39145123902276E-16));
#128517=DIRECTION('center_axis',(-0.310034691293285,-0.950725244291339,
-7.86457195103406E-6));
#128518=DIRECTION('ref_axis',(-3.83082999767964E-6,-7.02293516957875E-6,
0.999999999968002));
#128519=DIRECTION('center_axis',(0.405758682640086,0.913980246723271,-7.86457225038894E-6));
#128520=DIRECTION('ref_axis',(0.775097908773516,-0.344097741585796,0.52992450033045));
#128521=DIRECTION('center_axis',(-1.4081690688991E-16,-6.98296267768627E-15,
1.));
#128522=DIRECTION('ref_axis',(-1.,8.07722881720021E-31,-1.42096112075504E-16));
#128523=DIRECTION('center_axis',(-0.309991330356945,-0.950739383326507,
9.77058572337612E-6));
#128524=DIRECTION('ref_axis',(0.831557796518639,-0.271126846795441,0.484769908302721));
#128525=DIRECTION('center_axis',(0.405800366992264,0.913961739928691,9.77051586747459E-6));
#128526=DIRECTION('ref_axis',(0.799394020104308,-0.354937311790024,0.4847563360295));
#128527=DIRECTION('center_axis',(-1.4081690688991E-16,-6.98296267768627E-15,
1.));
#128528=DIRECTION('ref_axis',(-1.,8.24049048117772E-31,-1.37719829560012E-16));
#128529=DIRECTION('center_axis',(0.306544809307919,0.951856228406631,-1.81624797016104E-5));
#128530=DIRECTION('ref_axis',(0.82358590198436,-0.265244982896167,-0.501349539843232));
#128531=DIRECTION('center_axis',(-0.409108930222424,-0.912485552150557,
-1.81316453007737E-5));
#128532=DIRECTION('ref_axis',(0.791111768376538,-0.35468161961952,-0.498340364249396));
#128533=DIRECTION('center_axis',(-1.4081690688991E-16,-6.98296267768627E-15,
1.));
#128534=DIRECTION('ref_axis',(-1.,8.26087817385229E-31,-1.38060560438432E-16));
#128535=DIRECTION('center_axis',(0.306531947828316,0.95186037033724,-1.84940663645596E-5));
#128536=DIRECTION('ref_axis',(0.825248669207167,-0.265748920299591,0.498339387698185));
#128537=DIRECTION('center_axis',(-0.409121259236094,-0.912480024382929,
-1.85256990525701E-5));
#128538=DIRECTION('ref_axis',(0.789515382129796,-0.35399877972475,0.50134850686307));
#128539=DIRECTION('center_axis',(-1.4081690688991E-16,-6.98296267768627E-15,
1.));
#128540=DIRECTION('ref_axis',(-1.,9.83319205199467E-31,-1.40816906889911E-16));
#128541=DIRECTION('center_axis',(-1.4081690688991E-16,-6.98296267768627E-15,
1.));
#128542=DIRECTION('ref_axis',(-1.,8.46073526001725E-31,-1.4081690688991E-16));
#128543=DIRECTION('',(-0.913545457642603,0.406736643075795,2.71158415259712E-15));
#128544=DIRECTION('center_axis',(-1.4081690688991E-16,-6.98296267768627E-15,
1.));
#128545=DIRECTION('ref_axis',(-1.,7.97077743482043E-31,-1.4081690688991E-16));
#128546=DIRECTION('center_axis',(-1.4081690688991E-16,-6.98296267768627E-15,
1.));
#128547=DIRECTION('ref_axis',(-1.,7.97077743482043E-31,-1.4081690688991E-16));
#128548=DIRECTION('center_axis',(-1.4081690688991E-16,-6.98296267768627E-15,
1.));
#128549=DIRECTION('ref_axis',(-1.,7.97077743482043E-31,-1.4081690688991E-16));
#128550=DIRECTION('',(0.866025403784442,-0.499999999999995,-3.36953032019409E-15));
#128551=DIRECTION('center_axis',(1.4081690688991E-16,6.98296267768627E-15,
-1.));
#128552=DIRECTION('ref_axis',(1.,-7.97077743482043E-31,1.4081690688991E-16));
#128553=DIRECTION('',(-0.456779414654135,0.203366068089035,-0.866022406579779));
#128554=DIRECTION('center_axis',(1.4081690688991E-16,6.98296267768627E-15,
-1.));
#128555=DIRECTION('ref_axis',(-1.,7.97577417048809E-31,-1.40816906889911E-16));
#128556=DIRECTION('',(0.433014808647741,-0.250006733496384,0.866022406579777));
#128557=DIRECTION('center_axis',(-1.4081690688991E-16,-6.98296267768627E-15,
1.));
#128558=DIRECTION('ref_axis',(-1.,9.83319205199467E-31,-1.40816906889911E-16));
#128559=DIRECTION('center_axis',(-1.4081690688991E-16,-6.98296267768627E-15,
1.));
#128560=DIRECTION('ref_axis',(-1.,7.98248735348668E-31,-1.4081690688991E-16));
#128561=DIRECTION('',(-0.913545457642603,0.406736643075795,2.71158415259712E-15));
#128562=DIRECTION('center_axis',(1.4081690688991E-16,6.98296267768627E-15,
-1.));
#128563=DIRECTION('ref_axis',(-1.,-8.88178419700125E-16,-1.40816906889917E-16));
#128564=DIRECTION('',(0.866025403784442,-0.499999999999995,-3.36953032019409E-15));
#128565=DIRECTION('center_axis',(-1.4081690688991E-16,-6.98296267768627E-15,
1.));
#128566=DIRECTION('ref_axis',(-1.,7.99150043815584E-31,-1.4081690688991E-16));
#128567=DIRECTION('center_axis',(-1.4081690688991E-16,-6.98296267768627E-15,
1.));
#128568=DIRECTION('ref_axis',(1.,-7.99370576998456E-31,1.4081690688991E-16));
#128569=DIRECTION('',(-0.456775406784115,0.203374579494968,0.866022521746664));
#128570=DIRECTION('center_axis',(-1.4081690688991E-16,-6.98296267768627E-15,
1.));
#128571=DIRECTION('ref_axis',(-1.,7.99858039355471E-31,-1.4081690688991E-16));
#128572=DIRECTION('center_axis',(-1.4081690688991E-16,-6.98296267768627E-15,
1.));
#128573=DIRECTION('ref_axis',(-1.,7.99858039355471E-31,-1.4081690688991E-16));
#128574=DIRECTION('center_axis',(-1.4081690688991E-16,-6.98296267768627E-15,
1.));
#128575=DIRECTION('ref_axis',(-1.,7.99858039355471E-31,-1.4081690688991E-16));
#128576=DIRECTION('',(0.433019338752905,-0.249998488182556,-0.866022521746654));
#128577=DIRECTION('center_axis',(-1.4081690688991E-16,-6.98296267768627E-15,
1.));
#128578=DIRECTION('ref_axis',(-1.,9.83319205199467E-31,-1.40816906889911E-16));
#128579=DIRECTION('',(-0.913545457642603,0.406736643075795,2.71158415259712E-15));
#128580=DIRECTION('center_axis',(1.4081690688991E-16,6.98296267768627E-15,
-1.));
#128581=DIRECTION('ref_axis',(-1.,-8.88178419700124E-16,-1.40816906889917E-16));
#128582=DIRECTION('',(0.866025403784442,-0.499999999999995,-3.36953032019409E-15));
#128583=DIRECTION('center_axis',(-1.4081690688991E-16,-6.98296267768627E-15,
1.));
#128584=DIRECTION('ref_axis',(-1.,8.32577322149061E-31,-1.39145123902276E-16));
#128585=DIRECTION('center_axis',(-0.40771413759047,-0.913109622086531,-7.86457197304049E-6));
#128586=DIRECTION('ref_axis',(-4.54394094117637E-6,-6.58403204443663E-6,
0.999999999968002));
#128587=DIRECTION('center_axis',(0.499072844768338,0.866560035746507,-7.86457221234716E-6));
#128588=DIRECTION('ref_axis',(0.734883833187562,-0.42323253143994,0.529924500330467));
#128589=DIRECTION('center_axis',(-1.4081690688991E-16,-6.98296267768627E-15,
1.));
#128590=DIRECTION('ref_axis',(-1.,8.07722881720021E-31,-1.42096112075504E-16));
#128591=DIRECTION('center_axis',(-0.407672492120118,-0.913128216119242,
9.77058304390627E-6));
#128592=DIRECTION('ref_axis',(0.798661963253854,-0.356563044147659,0.484769908306667));
#128593=DIRECTION('center_axis',(0.499112366281669,0.866537273133274,9.77051750932866E-6));
#128594=DIRECTION('ref_axis',(0.75791380426364,-0.436552356525874,0.484756336027001));
#128595=DIRECTION('center_axis',(-1.4081690688991E-16,-6.98296267768627E-15,
1.));
#128596=DIRECTION('ref_axis',(-1.,8.24049048117772E-31,-1.37719829560012E-16));
#128597=DIRECTION('center_axis',(0.404361593575304,0.914599202553427,-1.81624796427904E-5));
#128598=DIRECTION('ref_axis',(0.791348561789414,-0.349880111830527,-0.5013495398415));
#128599=DIRECTION('center_axis',(-0.50224850121709,-0.864723333035735,-1.81316452500637E-5));
#128600=DIRECTION('ref_axis',(0.749703650682099,-0.435432334015447,-0.498340364256994));
#128601=DIRECTION('center_axis',(-1.4081690688991E-16,-6.98296267768627E-15,
1.));
#128602=DIRECTION('ref_axis',(-1.,8.26087817385229E-31,-1.38060560438432E-16));
#128603=DIRECTION('center_axis',(0.404349235502748,0.914604666184419,-1.84940679887669E-5));
#128604=DIRECTION('ref_axis',(0.792949544396104,-0.350555095114341,0.498339387698169));
#128605=DIRECTION('center_axis',(-0.502260184873573,-0.864716546821883,
-1.8525716205892E-5));
#128606=DIRECTION('ref_axis',(0.748187385815693,-0.434586366990651,0.501348506861391));
#128607=DIRECTION('center_axis',(-1.4081690688991E-16,-6.98296267768627E-15,
1.));
#128608=DIRECTION('ref_axis',(-1.,9.83319205199467E-31,-1.40816906889911E-16));
#128609=DIRECTION('center_axis',(-1.4081690688991E-16,-6.98296267768627E-15,
1.));
#128610=DIRECTION('ref_axis',(-1.,8.46073526001725E-31,-1.4081690688991E-16));
#128611=DIRECTION('',(-0.866025403784442,0.499999999999995,3.36953032019409E-15));
#128612=DIRECTION('center_axis',(-1.4081690688991E-16,-6.98296267768627E-15,
1.));
#128613=DIRECTION('ref_axis',(-1.,7.97077743482043E-31,-1.4081690688991E-16));
#128614=DIRECTION('center_axis',(-1.4081690688991E-16,-6.98296267768627E-15,
1.));
#128615=DIRECTION('ref_axis',(-1.,7.97077743482043E-31,-1.4081690688991E-16));
#128616=DIRECTION('center_axis',(-1.4081690688991E-16,-6.98296267768627E-15,
1.));
#128617=DIRECTION('ref_axis',(-1.,7.97077743482043E-31,-1.4081690688991E-16));
#128618=DIRECTION('',(0.80901699437495,-0.587785252292469,-3.99055920848346E-15));
#128619=DIRECTION('center_axis',(1.4081690688991E-16,6.98296267768627E-15,
-1.));
#128620=DIRECTION('ref_axis',(1.,-7.97077743482043E-31,1.4081690688991E-16));
#128621=DIRECTION('',(-0.433019586648885,0.249998457755584,-0.866022406579794));
#128622=DIRECTION('center_axis',(1.4081690688991E-16,6.98296267768627E-15,
-1.));
#128623=DIRECTION('ref_axis',(-1.,7.97577417048809E-31,-1.40816906889911E-16));
#128624=DIRECTION('',(0.404509888559933,-0.293899542971735,0.866022406579781));
#128625=DIRECTION('center_axis',(-1.4081690688991E-16,-6.98296267768627E-15,
1.));
#128626=DIRECTION('ref_axis',(-1.,9.83319205199467E-31,-1.40816906889911E-16));
#128627=DIRECTION('center_axis',(-1.4081690688991E-16,-6.98296267768627E-15,
1.));
#128628=DIRECTION('ref_axis',(-1.,7.98248735348668E-31,-1.4081690688991E-16));
#128629=DIRECTION('',(-0.866025403784442,0.499999999999995,3.36953032019409E-15));
#128630=DIRECTION('center_axis',(1.4081690688991E-16,6.98296267768627E-15,
-1.));
#128631=DIRECTION('ref_axis',(-1.,-8.88178419700125E-16,-1.40816906889917E-16));
#128632=DIRECTION('',(0.80901699437495,-0.587785252292469,-3.99055920848346E-15));
#128633=DIRECTION('center_axis',(-1.4081690688991E-16,-6.98296267768627E-15,
1.));
#128634=DIRECTION('ref_axis',(-1.,7.99150043815584E-31,-1.4081690688991E-16));
#128635=DIRECTION('center_axis',(-1.4081690688991E-16,-6.98296267768627E-15,
1.));
#128636=DIRECTION('ref_axis',(1.,-7.99370576998456E-31,1.4081690688991E-16));
#128637=DIRECTION('',(-0.433014711050232,0.250006503598672,0.866022521746664));
#128638=DIRECTION('center_axis',(-1.4081690688991E-16,-6.98296267768627E-15,
1.));
#128639=DIRECTION('ref_axis',(-1.,7.99858039355471E-31,-1.4081690688991E-16));
#128640=DIRECTION('center_axis',(-1.4081690688991E-16,-6.98296267768627E-15,
1.));
#128641=DIRECTION('ref_axis',(-1.,7.99858039355471E-31,-1.4081690688991E-16));
#128642=DIRECTION('center_axis',(-1.4081690688991E-16,-6.98296267768627E-15,
1.));
#128643=DIRECTION('ref_axis',(-1.,7.99858039355471E-31,-1.4081690688991E-16));
#128644=DIRECTION('',(0.4045152557187,-0.293891816351548,-0.866022521746648));
#128645=DIRECTION('center_axis',(-1.4081690688991E-16,-6.98296267768627E-15,
1.));
#128646=DIRECTION('ref_axis',(-1.,9.83319205199467E-31,-1.40816906889911E-16));
#128647=DIRECTION('',(-0.866025403784442,0.499999999999995,3.36953032019409E-15));
#128648=DIRECTION('center_axis',(1.4081690688991E-16,6.98296267768627E-15,
-1.));
#128649=DIRECTION('ref_axis',(-1.,8.01265634860448E-31,-1.4081690688991E-16));
#128650=DIRECTION('',(0.80901699437495,-0.587785252292469,-3.99055920848346E-15));
#128651=DIRECTION('center_axis',(-1.4081690688991E-16,-6.98296267768627E-15,
1.));
#128652=DIRECTION('ref_axis',(-1.,8.32577322149061E-31,-1.39145123902276E-16));
#128653=DIRECTION('center_axis',(-0.500926582476549,-0.865489779781664,
-7.86457205664364E-6));
#128654=DIRECTION('ref_axis',(-5.20726753510821E-6,-6.0729929450695E-6,
0.999999999968002));
#128655=DIRECTION('center_axis',(0.586919060371537,0.809645611678802,-7.86457238663011E-6));
#128656=DIRECTION('ref_axis',(0.686618216540999,-0.497730297112391,0.529924500330442));
#128657=DIRECTION('center_axis',(-1.4081690688991E-16,-6.98296267768627E-15,
1.));
#128658=DIRECTION('ref_axis',(-1.,8.07722881720021E-31,-1.42096112075504E-16));
#128659=DIRECTION('center_axis',(-0.500887108752324,-0.865512625090052,
9.77058776453254E-6));
#128660=DIRECTION('ref_axis',(0.757015822392177,-0.438092662173928,0.484769908304193));
#128661=DIRECTION('center_axis',(0.586955986040212,0.809618842638991,9.77051913842785E-6));
#128662=DIRECTION('ref_axis',(0.708129726178395,-0.513384442288506,0.484756336027318));
#128663=DIRECTION('center_axis',(-1.4081690688991E-16,-6.98296267768627E-15,
1.));
#128664=DIRECTION('ref_axis',(-1.,8.24049048117772E-31,-1.37719829560012E-16));
#128665=DIRECTION('center_axis',(0.497748107605313,0.867321636444897,-1.8162479830695E-5));
#128666=DIRECTION('ref_axis',(0.750441041151826,-0.430681881043238,-0.501349539838247));
#128667=DIRECTION('center_axis',(-0.58988533253017,-0.807487024129189,-1.81316452233006E-5));
#128668=DIRECTION('ref_axis',(0.700081622911622,-0.51141236064337,-0.498340364251789));
#128669=DIRECTION('center_axis',(-1.4081690688991E-16,-6.98296267768627E-15,
1.));
#128670=DIRECTION('ref_axis',(-1.,8.26087817385229E-31,-1.38060560438432E-16));
#128671=DIRECTION('center_axis',(0.497736388334897,0.867328361916813,-1.84940646400988E-5));
#128672=DIRECTION('ref_axis',(0.751962698442603,-0.431520514949369,0.498339387695524));
#128673=DIRECTION('center_axis',(-0.589896242825295,-0.807479053819601,
-1.85257260569587E-5));
#128674=DIRECTION('ref_axis',(0.698662091935,-0.510412535077464,0.50134850685806));
#128675=DIRECTION('center_axis',(-1.4081690688991E-16,-6.98296267768627E-15,
1.));
#128676=DIRECTION('ref_axis',(-1.,9.83319205199467E-31,-1.40816906889911E-16));
#128677=DIRECTION('center_axis',(-1.4081690688991E-16,-6.98296267768627E-15,
1.));
#128678=DIRECTION('ref_axis',(-1.,8.46073526001725E-31,-1.4081690688991E-16));
#128679=DIRECTION('',(-0.80901699437495,0.587785252292469,3.99055920848346E-15));
#128680=DIRECTION('center_axis',(-1.4081690688991E-16,-6.98296267768627E-15,
1.));
#128681=DIRECTION('ref_axis',(-1.,7.97077743482043E-31,-1.4081690688991E-16));
#128682=DIRECTION('center_axis',(-1.4081690688991E-16,-6.98296267768627E-15,
1.));
#128683=DIRECTION('ref_axis',(-1.,7.97077743482043E-31,-1.4081690688991E-16));
#128684=DIRECTION('center_axis',(-1.4081690688991E-16,-6.98296267768627E-15,
1.));
#128685=DIRECTION('ref_axis',(-1.,7.97077743482043E-31,-1.4081690688991E-16));
#128686=DIRECTION('',(0.743144825477398,-0.669130606358854,-4.56786669500649E-15));
#128687=DIRECTION('center_axis',(1.4081690688991E-16,6.98296267768627E-15,
-1.));
#128688=DIRECTION('ref_axis',(1.,-7.97077743482043E-31,1.4081690688991E-16));
#128689=DIRECTION('',(-0.404515505437171,0.293891812003427,-0.866022406579791));
#128690=DIRECTION('center_axis',(1.4081690688991E-16,6.98296267768627E-15,
-1.));
#128691=DIRECTION('ref_axis',(-1.,-8.88178419700124E-16,-1.40816906889917E-16));
#128692=DIRECTION('',(0.371573073483921,-0.33457232755186,0.866022406579786));
#128693=DIRECTION('center_axis',(-1.4081690688991E-16,-6.98296267768627E-15,
1.));
#128694=DIRECTION('ref_axis',(-1.,9.83319205199467E-31,-1.40816906889911E-16));
#128695=DIRECTION('center_axis',(-1.4081690688991E-16,-6.98296267768627E-15,
1.));
#128696=DIRECTION('ref_axis',(-1.,7.98248735348668E-31,-1.4081690688991E-16));
#128697=DIRECTION('',(-0.80901699437495,0.587785252292469,3.99055920848346E-15));
#128698=DIRECTION('center_axis',(1.4081690688991E-16,6.98296267768627E-15,
-1.));
#128699=DIRECTION('ref_axis',(-1.,7.98707387273907E-31,-1.4081690688991E-16));
#128700=DIRECTION('',(0.743144825477398,-0.669130606358854,-4.56786669500649E-15));
#128701=DIRECTION('center_axis',(-1.4081690688991E-16,-6.98296267768627E-15,
1.));
#128702=DIRECTION('ref_axis',(-1.,7.99150043815584E-31,-1.4081690688991E-16));
#128703=DIRECTION('center_axis',(-1.4081690688991E-16,-6.98296267768627E-15,
1.));
#128704=DIRECTION('ref_axis',(1.,-7.99370576998456E-31,1.4081690688991E-16));
#128705=DIRECTION('',(-0.404509815527948,0.293899304131707,0.86602252174666));
#128706=DIRECTION('center_axis',(-1.4081690688991E-16,-6.98296267768627E-15,
1.));
#128707=DIRECTION('ref_axis',(-1.,7.99858039355471E-31,-1.4081690688991E-16));
#128708=DIRECTION('center_axis',(-1.4081690688991E-16,-6.98296267768627E-15,
1.));
#128709=DIRECTION('ref_axis',(-1.,7.99858039355471E-31,-1.4081690688991E-16));
#128710=DIRECTION('center_axis',(-1.4081690688991E-16,-6.98296267768627E-15,
1.));
#128711=DIRECTION('ref_axis',(-1.,7.99858039355471E-31,-1.4081690688991E-16));
#128712=DIRECTION('',(0.371579218892551,-0.33456520427975,-0.866022521746664));
#128713=DIRECTION('center_axis',(-1.4081690688991E-16,-6.98296267768627E-15,
1.));
#128714=DIRECTION('ref_axis',(-1.,9.83319205199467E-31,-1.40816906889911E-16));
#128715=DIRECTION('',(-0.80901699437495,0.587785252292469,3.99055920848346E-15));
#128716=DIRECTION('center_axis',(1.4081690688991E-16,6.98296267768627E-15,
-1.));
#128717=DIRECTION('ref_axis',(-1.,8.01265634860448E-31,-1.4081690688991E-16));
#128718=DIRECTION('',(0.743144825477398,-0.669130606358854,-4.56786669500649E-15));
#128719=DIRECTION('center_axis',(-1.4081690688991E-16,-6.98296267768627E-15,
1.));
#128720=DIRECTION('ref_axis',(-1.,8.32577322149061E-31,-1.39145123902276E-16));
#128721=DIRECTION('center_axis',(-0.588650770899369,-0.808387450334138,
-7.86457204757439E-6));
#128722=DIRECTION('ref_axis',(-5.81354223910265E-6,-5.4954167425029E-6,
0.999999999968001));
#128723=DIRECTION('center_axis',(0.668334867928669,0.743860540860259,-7.8645723350969E-6));
#128724=DIRECTION('ref_axis',(0.630829867029799,-0.566774825493072,0.529924500330438));
#128725=DIRECTION('center_axis',(-1.4081690688991E-16,-6.98296267768627E-15,
1.));
#128726=DIRECTION('ref_axis',(-1.,8.07722881720021E-31,-1.42096112075504E-16));
#128727=DIRECTION('center_axis',(-0.588613901400178,-0.808414296622096,
9.77058519236102E-6));
#128728=DIRECTION('ref_axis',(0.707075657763138,-0.514822445315961,0.484769908304672));
#128729=DIRECTION('center_axis',(0.668368793191875,0.743830058677232,9.77050991880942E-6));
#128730=DIRECTION('ref_axis',(0.650587230628311,-0.584591780669575,0.484756336025596));
#128731=DIRECTION('center_axis',(-1.4081690688991E-16,-6.98296267768627E-15,
1.));
#128732=DIRECTION('ref_axis',(-1.,8.24049048117772E-31,-1.37719829560012E-16));
#128733=DIRECTION('center_axis',(0.58568118920789,0.81054151298879,-1.81624800754865E-5));
#128734=DIRECTION('ref_axis',(0.70131153142444,-0.506765009439537,-0.50134953984107));
#128735=DIRECTION('center_axis',(-0.671059256698626,-0.741403718408757,
-1.81316452525126E-5));
#128736=DIRECTION('ref_axis',(0.642789354378864,-0.58178924642884,-0.49834036424613));
#128737=DIRECTION('center_axis',(-1.4081690688991E-16,-6.98296267768627E-15,
1.));
#128738=DIRECTION('ref_axis',(-1.,8.26087817385229E-31,-1.38060560438432E-16));
#128739=DIRECTION('center_axis',(0.585670237127502,0.810549426624303,-1.84940374120092E-5));
#128740=DIRECTION('ref_axis',(0.702737191803893,-0.507758105719546,0.49833938769846));
#128741=DIRECTION('center_axis',(-0.671069274109347,-0.741394651318144,
-1.85257084724781E-5));
#128742=DIRECTION('ref_axis',(0.641482109966384,-0.580646516615919,0.501348506864113));
#128743=DIRECTION('center_axis',(-1.4081690688991E-16,-6.98296267768627E-15,
1.));
#128744=DIRECTION('ref_axis',(-1.,9.83319205199467E-31,-1.40816906889911E-16));
#128745=DIRECTION('center_axis',(-1.4081690688991E-16,-6.98296267768627E-15,
1.));
#128746=DIRECTION('ref_axis',(-1.,8.46073526001725E-31,-1.4081690688991E-16));
#128747=DIRECTION('',(-0.743144825477398,0.669130606358854,4.56786669500649E-15));
#128748=DIRECTION('center_axis',(-1.4081690688991E-16,-6.98296267768627E-15,
1.));
#128749=DIRECTION('ref_axis',(-1.,7.97077743482043E-31,-1.4081690688991E-16));
#128750=DIRECTION('center_axis',(-1.4081690688991E-16,-6.98296267768627E-15,
1.));
#128751=DIRECTION('ref_axis',(-1.,7.97077743482043E-31,-1.4081690688991E-16));
#128752=DIRECTION('center_axis',(-1.4081690688991E-16,-6.98296267768627E-15,
1.));
#128753=DIRECTION('ref_axis',(-1.,7.97077743482043E-31,-1.4081690688991E-16));
#128754=DIRECTION('',(0.669130606358862,-0.743144825477391,-5.09512767813147E-15));
#128755=DIRECTION('center_axis',(1.4081690688991E-16,6.98296267768627E-15,
-1.));
#128756=DIRECTION('ref_axis',(1.,-7.97077743482043E-31,1.4081690688991E-16));
#128757=DIRECTION('',(-0.371579467697567,0.33456522605815,-0.86602240657979));
#128758=DIRECTION('center_axis',(1.4081690688991E-16,6.98296267768627E-15,
-1.));
#128759=DIRECTION('ref_axis',(-1.,8.88178419700126E-16,-1.40816906889904E-16));
#128760=DIRECTION('',(0.334565226058153,-0.371579467697543,0.866022406579799));
#128761=DIRECTION('center_axis',(-1.4081690688991E-16,-6.98296267768627E-15,
1.));
#128762=DIRECTION('ref_axis',(-1.,9.83319205199467E-31,-1.40816906889911E-16));
#128763=DIRECTION('center_axis',(-1.4081690688991E-16,-6.98296267768627E-15,
1.));
#128764=DIRECTION('ref_axis',(-1.,7.98248735348668E-31,-1.4081690688991E-16));
#128765=DIRECTION('',(-0.743144825477398,0.669130606358854,4.56786669500649E-15));
#128766=DIRECTION('center_axis',(1.4081690688991E-16,6.98296267768627E-15,
-1.));
#128767=DIRECTION('ref_axis',(-1.,7.98707387273907E-31,-1.4081690688991E-16));
#128768=DIRECTION('',(0.669130606358862,-0.743144825477391,-5.09512767813147E-15));
#128769=DIRECTION('center_axis',(-1.4081690688991E-16,-6.98296267768627E-15,
1.));
#128770=DIRECTION('ref_axis',(-1.,7.99150043815584E-31,-1.4081690688991E-16));
#128771=DIRECTION('center_axis',(-1.4081690688991E-16,-6.98296267768627E-15,
1.));
#128772=DIRECTION('ref_axis',(1.,-7.99370576998456E-31,1.4081690688991E-16));
#128773=DIRECTION('',(-0.3715730258176,0.334572082386297,0.866022521746663));
#128774=DIRECTION('center_axis',(-1.4081690688991E-16,-6.98296267768627E-15,
1.));
#128775=DIRECTION('ref_axis',(-1.,7.99858039355471E-31,-1.4081690688991E-16));
#128776=DIRECTION('center_axis',(-1.4081690688991E-16,-6.98296267768627E-15,
1.));
#128777=DIRECTION('ref_axis',(-1.,7.99858039355471E-31,-1.4081690688991E-16));
#128778=DIRECTION('center_axis',(-1.4081690688991E-16,-6.98296267768627E-15,
1.));
#128779=DIRECTION('ref_axis',(-1.,7.99858039355471E-31,-1.4081690688991E-16));
#128780=DIRECTION('',(0.334572082386317,-0.37157302581762,-0.866022521746647));
#128781=DIRECTION('center_axis',(-1.4081690688991E-16,-6.98296267768627E-15,
1.));
#128782=DIRECTION('ref_axis',(-1.,9.83319205199467E-31,-1.40816906889911E-16));
#128783=DIRECTION('',(-0.743144825477398,0.669130606358854,4.56786669500649E-15));
#128784=DIRECTION('center_axis',(1.4081690688991E-16,6.98296267768627E-15,
-1.));
#128785=DIRECTION('ref_axis',(-1.,8.88178419700126E-16,-1.40816906889904E-16));
#128786=DIRECTION('',(0.669130606358862,-0.743144825477391,-5.09512767813147E-15));
#128787=DIRECTION('center_axis',(-1.4081690688991E-16,-6.98296267768627E-15,
1.));
#128788=DIRECTION('ref_axis',(-1.,8.32577322149061E-31,-1.39145123902276E-16));
#128789=DIRECTION('center_axis',(-0.669925578293101,-0.742428258814818,
-7.86457203518997E-6));
#128790=DIRECTION('ref_axis',(-6.35612246172978E-6,-4.85763167245441E-6,
0.999999999968002));
#128791=DIRECTION('center_axis',(0.742428258814711,0.66992557829322,-7.86457232381813E-6));
#128792=DIRECTION('ref_axis',(0.568130013485777,-0.629609650280374,0.529924500330449));
#128793=DIRECTION('center_axis',(-1.4081690688991E-16,-6.98296267768627E-15,
1.));
#128794=DIRECTION('ref_axis',(-1.,8.07722881720021E-31,-1.42096112075504E-16));
#128795=DIRECTION('center_axis',(-0.669891716968524,-0.742458811949524,
9.77058138072136E-6));
#128796=DIRECTION('ref_axis',(0.649388624263403,-0.585911726014202,0.484769908303252));
#128797=DIRECTION('center_axis',(0.742458811977019,0.669891716938052,9.77050718766635E-6));
#128798=DIRECTION('ref_axis',(0.585916765234264,-0.649394209167008,0.484756336026434));
#128799=DIRECTION('center_axis',(-1.4081690688991E-16,-6.98296267768627E-15,
1.));
#128800=DIRECTION('ref_axis',(-1.,8.24049048117772E-31,-1.37719829560012E-16));
#128801=DIRECTION('center_axis',(0.667197425140074,0.744880927099479,-1.8162479743951E-5));
#128802=DIRECTION('ref_axis',(0.644498305799933,-0.57729591434456,-0.501349539844304));
#128803=DIRECTION('center_axis',(-0.744880915222522,-0.667197438400734,
-1.81316451348809E-5));
#128804=DIRECTION('ref_axis',(0.578454551160941,-0.645791927477339,-0.498340364255494));
#128805=DIRECTION('center_axis',(-1.4081690688991E-16,-6.98296267768627E-15,
1.));
#128806=DIRECTION('ref_axis',(-1.,8.26087817385229E-31,-1.38060560438432E-16));
#128807=DIRECTION('center_axis',(0.667187360262395,0.74488994218211,-1.84940515154987E-5));
#128808=DIRECTION('ref_axis',(0.645812349436813,-0.578432592429817,0.498339387696602));
#128809=DIRECTION('center_axis',(-0.744889929984709,-0.667187373879462,
-1.85257164452763E-5));
#128810=DIRECTION('ref_axis',(0.577273915766496,-0.644518813413982,0.501348506860296));
#128811=DIRECTION('center_axis',(-1.4081690688991E-16,-6.98296267768627E-15,
1.));
#128812=DIRECTION('ref_axis',(-1.,9.83319205199467E-31,-1.40816906889911E-16));
#128813=DIRECTION('center_axis',(-1.4081690688991E-16,-6.98296267768627E-15,
1.));
#128814=DIRECTION('ref_axis',(-1.,8.46073526001725E-31,-1.4081690688991E-16));
#128815=DIRECTION('',(-0.669130606358862,0.743144825477391,5.09512767813147E-15));
#128816=DIRECTION('center_axis',(-1.4081690688991E-16,-6.98296267768627E-15,
1.));
#128817=DIRECTION('ref_axis',(-1.,7.97077743482043E-31,-1.4081690688991E-16));
#128818=DIRECTION('center_axis',(-1.4081690688991E-16,-6.98296267768627E-15,
1.));
#128819=DIRECTION('ref_axis',(-1.,7.97077743482043E-31,-1.4081690688991E-16));
#128820=DIRECTION('center_axis',(-1.4081690688991E-16,-6.98296267768627E-15,
1.));
#128821=DIRECTION('ref_axis',(-1.,7.97077743482043E-31,-1.4081690688991E-16));
#128822=DIRECTION('',(0.587785252292477,-0.809016994374945,-5.56656537619083E-15));
#128823=DIRECTION('center_axis',(1.4081690688991E-16,6.98296267768627E-15,
-1.));
#128824=DIRECTION('ref_axis',(1.,-7.97077743482043E-31,1.4081690688991E-16));
#128825=DIRECTION('',(-0.334572327551839,0.371573073483901,-0.866022406579803));
#128826=DIRECTION('center_axis',(1.4081690688991E-16,6.98296267768627E-15,
-1.));
#128827=DIRECTION('ref_axis',(-1.,8.88178419700126E-16,-1.40816906889904E-16));
#128828=DIRECTION('',(0.293891812003449,-0.404515505437191,0.866022406579774));
#128829=DIRECTION('center_axis',(-1.4081690688991E-16,-6.98296267768627E-15,
1.));
#128830=DIRECTION('ref_axis',(-1.,9.83319205199467E-31,-1.40816906889911E-16));
#128831=DIRECTION('center_axis',(-1.4081690688991E-16,-6.98296267768627E-15,
1.));
#128832=DIRECTION('ref_axis',(-1.,7.98248735348668E-31,-1.4081690688991E-16));
#128833=DIRECTION('',(-0.669130606358862,0.743144825477391,5.09512767813147E-15));
#128834=DIRECTION('center_axis',(1.4081690688991E-16,6.98296267768627E-15,
-1.));
#128835=DIRECTION('ref_axis',(-1.,7.98707387273907E-31,-1.4081690688991E-16));
#128836=DIRECTION('',(0.587785252292477,-0.809016994374945,-5.56656537619083E-15));
#128837=DIRECTION('center_axis',(-1.4081690688991E-16,-6.98296267768627E-15,
1.));
#128838=DIRECTION('ref_axis',(-1.,7.99150043815584E-31,-1.4081690688991E-16));
#128839=DIRECTION('center_axis',(-1.4081690688991E-16,-6.98296267768627E-15,
1.));
#128840=DIRECTION('ref_axis',(1.,-1.06581410364015E-14,1.40816906889836E-16));
#128841=DIRECTION('',(-0.334565204279747,0.371579218892574,0.866022521746655));
#128842=DIRECTION('center_axis',(-1.4081690688991E-16,-6.98296267768627E-15,
1.));
#128843=DIRECTION('ref_axis',(-1.,7.99858039355471E-31,-1.4081690688991E-16));
#128844=DIRECTION('center_axis',(-1.4081690688991E-16,-6.98296267768627E-15,
1.));
#128845=DIRECTION('ref_axis',(-1.,7.99858039355471E-31,-1.4081690688991E-16));
#128846=DIRECTION('center_axis',(-1.4081690688991E-16,-6.98296267768627E-15,
1.));
#128847=DIRECTION('ref_axis',(-1.,7.99858039355471E-31,-1.4081690688991E-16));
#128848=DIRECTION('',(0.293899304131692,-0.404509815527973,-0.866022521746654));
#128849=DIRECTION('center_axis',(-1.4081690688991E-16,-6.98296267768627E-15,
1.));
#128850=DIRECTION('ref_axis',(-1.,9.83319205199467E-31,-1.40816906889911E-16));
#128851=DIRECTION('',(-0.669130606358862,0.743144825477391,5.09512767813147E-15));
#128852=DIRECTION('center_axis',(1.4081690688991E-16,6.98296267768627E-15,
-1.));
#128853=DIRECTION('ref_axis',(-1.,8.01265634860448E-31,-1.4081690688991E-16));
#128854=DIRECTION('',(0.587785252292477,-0.809016994374945,-5.56656537619083E-15));
#128855=DIRECTION('center_axis',(-1.4081690688991E-16,-6.98296267768627E-15,
1.));
#128856=DIRECTION('ref_axis',(-1.,8.32577322149061E-31,-1.39145123902276E-16));
#128857=DIRECTION('center_axis',(-0.743860540860149,-0.668334867928791,
-7.86457203541079E-6));
#128858=DIRECTION('ref_axis',(-6.82906373999688E-6,-4.16662532737549E-6,
0.999999999968002));
#128859=DIRECTION('center_axis',(0.808387450334027,0.588650770899521,-7.86457235190628E-6));
#128860=DIRECTION('ref_axis',(0.499205608625243,-0.685546339984863,0.529924500330433));
#128861=DIRECTION('center_axis',(-1.4081690688991E-16,-6.98296267768627E-15,
1.));
#128862=DIRECTION('ref_axis',(-1.,8.07722881720021E-31,-1.42096112075504E-16));
#128863=DIRECTION('center_axis',(-0.74383005870373,-0.668368793162384,9.77058148516564E-6));
#128864=DIRECTION('ref_axis',(0.584586753102489,-0.6505816352322,0.484769908302574));
#128865=DIRECTION('center_axis',(0.808414296646392,0.58861390136681,9.7705106400194E-6));
#128866=DIRECTION('ref_axis',(0.514826873149565,-0.707081738814457,0.48475633602684));
#128867=DIRECTION('center_axis',(-1.4081690688991E-16,-6.98296267768627E-15,
1.));
#128868=DIRECTION('ref_axis',(-1.,8.24049048117772E-31,-1.37719829560012E-16));
#128869=DIRECTION('center_axis',(0.74140370646244,0.671059269896393,-1.81624792922045E-5));
#128870=DIRECTION('ref_axis',(0.580623821868732,-0.641501844406329,-0.501349539844034));
#128871=DIRECTION('center_axis',(-0.810541502562932,-0.585681203637498,
-1.81316452566355E-5));
#128872=DIRECTION('ref_axis',(0.507782078837387,-0.702719177034441,-0.498340364248792));
#128873=DIRECTION('center_axis',(-1.4081690688991E-16,-6.98296267768627E-15,
1.));
#128874=DIRECTION('ref_axis',(-1.,8.26087817385229E-31,-1.38060560438432E-16));
#128875=DIRECTION('center_axis',(0.74139463906873,0.671069287643322,-1.84940903563101E-5));
#128876=DIRECTION('ref_axis',(0.581811851822687,-0.642769650611083,0.498339387698746));
#128877=DIRECTION('center_axis',(-0.810549415911435,-0.585670251952778,
-1.85257190592093E-5));
#128878=DIRECTION('ref_axis',(0.506740987740971,-0.701329627215785,0.501348506861918));
#128879=DIRECTION('center_axis',(-1.4081690688991E-16,-6.98296267768627E-15,
1.));
#128880=DIRECTION('ref_axis',(-1.,9.83319205199467E-31,-1.40816906889911E-16));
#128881=DIRECTION('center_axis',(-1.4081690688991E-16,-6.98296267768627E-15,
1.));
#128882=DIRECTION('ref_axis',(-1.,8.46073526001725E-31,-1.4081690688991E-16));
#128883=DIRECTION('',(-0.587785252292477,0.809016994374945,5.56656537619083E-15));
#128884=DIRECTION('center_axis',(-1.4081690688991E-16,-6.98296267768627E-15,
1.));
#128885=DIRECTION('ref_axis',(-1.,7.97077743482043E-31,-1.4081690688991E-16));
#128886=DIRECTION('center_axis',(-1.4081690688991E-16,-6.98296267768627E-15,
1.));
#128887=DIRECTION('ref_axis',(-1.,7.97077743482043E-31,-1.4081690688991E-16));
#128888=DIRECTION('center_axis',(-1.4081690688991E-16,-6.98296267768627E-15,
1.));
#128889=DIRECTION('ref_axis',(-1.,7.97077743482043E-31,-1.4081690688991E-16));
#128890=DIRECTION('',(0.500000000000004,-0.866025403784436,-5.97701461910994E-15));
#128891=DIRECTION('center_axis',(1.4081690688991E-16,6.98296267768627E-15,
-1.));
#128892=DIRECTION('ref_axis',(1.,-7.97077743482043E-31,1.4081690688991E-16));
#128893=DIRECTION('',(-0.293899542971751,0.404509888559909,-0.866022406579787));
#128894=DIRECTION('center_axis',(1.4081690688991E-16,6.98296267768627E-15,
-1.));
#128895=DIRECTION('ref_axis',(-1.,7.97577417048809E-31,-1.40816906889911E-16));
#128896=DIRECTION('',(0.24999845775561,-0.433019586648882,0.866022406579788));
#128897=DIRECTION('center_axis',(-1.4081690688991E-16,-6.98296267768627E-15,
1.));
#128898=DIRECTION('ref_axis',(-1.,9.83319205199467E-31,-1.40816906889911E-16));
#128899=DIRECTION('center_axis',(-1.4081690688991E-16,-6.98296267768627E-15,
1.));
#128900=DIRECTION('ref_axis',(-1.,7.98248735348668E-31,-1.4081690688991E-16));
#128901=DIRECTION('',(-0.587785252292477,0.809016994374945,5.56656537619083E-15));
#128902=DIRECTION('center_axis',(1.4081690688991E-16,6.98296267768627E-15,
-1.));
#128903=DIRECTION('ref_axis',(-1.,-1.77635683940025E-15,-1.40816906889923E-16));
#128904=DIRECTION('',(0.500000000000004,-0.866025403784436,-5.97701461910994E-15));
#128905=DIRECTION('center_axis',(-1.4081690688991E-16,-6.98296267768627E-15,
1.));
#128906=DIRECTION('ref_axis',(-1.,7.99150043815584E-31,-1.4081690688991E-16));
#128907=DIRECTION('center_axis',(-1.4081690688991E-16,-6.98296267768627E-15,
1.));
#128908=DIRECTION('ref_axis',(1.,-1.06581410364015E-14,1.40816906889836E-16));
#128909=DIRECTION('',(-0.293891816351504,0.40451525571866,0.866022521746681));
#128910=DIRECTION('center_axis',(-1.4081690688991E-16,-6.98296267768627E-15,
1.));
#128911=DIRECTION('ref_axis',(-1.,7.99858039355471E-31,-1.4081690688991E-16));
#128912=DIRECTION('center_axis',(-1.4081690688991E-16,-6.98296267768627E-15,
1.));
#128913=DIRECTION('ref_axis',(-1.,7.99858039355471E-31,-1.4081690688991E-16));
#128914=DIRECTION('center_axis',(-1.4081690688991E-16,-6.98296267768627E-15,
1.));
#128915=DIRECTION('ref_axis',(-1.,7.99858039355471E-31,-1.4081690688991E-16));
#128916=DIRECTION('',(0.250006503598675,-0.43301471105021,-0.866022521746674));
#128917=DIRECTION('center_axis',(-1.4081690688991E-16,-6.98296267768627E-15,
1.));
#128918=DIRECTION('ref_axis',(-1.,9.83319205199467E-31,-1.40816906889911E-16));
#128919=DIRECTION('',(-0.587785252292477,0.809016994374945,5.56656537619083E-15));
#128920=DIRECTION('center_axis',(1.4081690688991E-16,6.98296267768627E-15,
-1.));
#128921=DIRECTION('ref_axis',(-1.,8.01265634860448E-31,-1.4081690688991E-16));
#128922=DIRECTION('',(0.500000000000004,-0.866025403784436,-5.97701461910994E-15));
#128923=DIRECTION('center_axis',(-1.4081690688991E-16,-6.98296267768627E-15,
1.));
#128924=DIRECTION('ref_axis',(-1.,8.32577322149061E-31,-1.39145123902276E-16));
#128925=DIRECTION('center_axis',(-0.809645611678698,-0.58691906037168,-7.86457201904425E-6));
#128926=DIRECTION('ref_axis',(-7.22718433787083E-6,-3.42996857467424E-6,
0.999999999968002));
#128927=DIRECTION('center_axis',(0.865489779781569,0.500926582476713,-7.86457233244357E-6));
#128928=DIRECTION('ref_axis',(0.424811802651058,-0.73397204052872,0.529924500330439));
#128929=DIRECTION('center_axis',(-1.4081690688991E-16,-6.98296267768627E-15,
1.));
#128930=DIRECTION('ref_axis',(-1.,8.07722881720021E-31,-1.42096112075504E-16));
#128931=DIRECTION('center_axis',(-0.809618842664134,-0.58695598600553,9.77059657011212E-6));
#128932=DIRECTION('ref_axis',(0.513380027140978,-0.708123635910311,0.484769908304848));
#128933=DIRECTION('center_axis',(0.86551262510965,0.50088710871846,9.77051708363798E-6));
#128934=DIRECTION('ref_axis',(0.438096430108474,-0.757022332965543,0.484756336026273));
#128935=DIRECTION('center_axis',(-1.4081690688991E-16,-6.98296267768627E-15,
1.));
#128936=DIRECTION('ref_axis',(-1.,8.24049048117772E-31,-1.37719829560012E-16));
#128937=DIRECTION('center_axis',(0.807487013627704,0.58988534690458,-1.81624797733012E-5));
#128938=DIRECTION('ref_axis',(0.51038790184082,-0.698679346016538,-0.50134953984663));
#128939=DIRECTION('center_axis',(-0.867321627584508,-0.497748123045586,
-1.81316451898425E-5));
#128940=DIRECTION('ref_axis',(0.431546239795072,-0.751947288231341,-0.498340364249442));
#128941=DIRECTION('center_axis',(-1.4081690688991E-16,-6.98296267768627E-15,
1.));
#128942=DIRECTION('ref_axis',(-1.,8.26087817385229E-31,-1.38060560438432E-16));
#128943=DIRECTION('center_axis',(0.807479043032716,0.589896257591909,-1.84940513261902E-5));
#128944=DIRECTION('ref_axis',(0.511436901809379,-0.700064389993352,0.498339387697642));
#128945=DIRECTION('center_axis',(-0.867328352822391,-0.497736404181166,
-1.85257110601528E-5));
#128946=DIRECTION('ref_axis',(0.430656099412309,-0.750456526860381,0.501348506860876));
#128947=DIRECTION('center_axis',(-1.4081690688991E-16,-6.98296267768627E-15,
1.));
#128948=DIRECTION('ref_axis',(-1.,9.83319205199467E-31,-1.40816906889911E-16));
#128949=DIRECTION('center_axis',(-1.4081690688991E-16,-6.98296267768627E-15,
1.));
#128950=DIRECTION('ref_axis',(-1.,8.46073526001725E-31,-1.4081690688991E-16));
#128951=DIRECTION('',(-0.500000000000004,0.866025403784436,5.97701461910994E-15));
#128952=DIRECTION('center_axis',(-1.4081690688991E-16,-6.98296267768627E-15,
1.));
#128953=DIRECTION('ref_axis',(-1.,7.97077743482043E-31,-1.4081690688991E-16));
#128954=DIRECTION('center_axis',(-1.4081690688991E-16,-6.98296267768627E-15,
1.));
#128955=DIRECTION('ref_axis',(-1.,7.97077743482043E-31,-1.4081690688991E-16));
#128956=DIRECTION('center_axis',(-1.4081690688991E-16,-6.98296267768627E-15,
1.));
#128957=DIRECTION('ref_axis',(-1.,7.97077743482043E-31,-1.4081690688991E-16));
#128958=DIRECTION('',(0.406736643075804,-0.913545457642599,-6.32197843909137E-15));
#128959=DIRECTION('center_axis',(1.4081690688991E-16,6.98296267768627E-15,
-1.));
#128960=DIRECTION('ref_axis',(1.,-7.97077743482043E-31,1.4081690688991E-16));
#128961=DIRECTION('',(-0.250006733496394,0.433014808647735,-0.866022406579777));
#128962=DIRECTION('center_axis',(1.4081690688991E-16,6.98296267768627E-15,
-1.));
#128963=DIRECTION('ref_axis',(-1.,7.97577417048809E-31,-1.40816906889911E-16));
#128964=DIRECTION('',(0.203366068089048,-0.456779414654134,0.866022406579776));
#128965=DIRECTION('center_axis',(-1.4081690688991E-16,-6.98296267768627E-15,
1.));
#128966=DIRECTION('ref_axis',(-1.,9.83319205199467E-31,-1.40816906889911E-16));
#128967=DIRECTION('center_axis',(-1.4081690688991E-16,-6.98296267768627E-15,
1.));
#128968=DIRECTION('ref_axis',(-1.,7.98248735348668E-31,-1.4081690688991E-16));
#128969=DIRECTION('',(-0.500000000000004,0.866025403784436,5.97701461910994E-15));
#128970=DIRECTION('center_axis',(1.4081690688991E-16,6.98296267768627E-15,
-1.));
#128971=DIRECTION('ref_axis',(-1.,7.98707387273907E-31,-1.4081690688991E-16));
#128972=DIRECTION('',(0.406736643075804,-0.913545457642599,-6.32197843909137E-15));
#128973=DIRECTION('center_axis',(-1.4081690688991E-16,-6.98296267768627E-15,
1.));
#128974=DIRECTION('ref_axis',(-1.,7.99150043815584E-31,-1.4081690688991E-16));
#128975=DIRECTION('center_axis',(-1.4081690688991E-16,-6.98296267768627E-15,
1.));
#128976=DIRECTION('ref_axis',(1.,4.44089209850062E-15,1.40816906889941E-16));
#128977=DIRECTION('',(-0.249998488182552,0.433019338752927,0.866022521746644));
#128978=DIRECTION('center_axis',(-1.4081690688991E-16,-6.98296267768627E-15,
1.));
#128979=DIRECTION('ref_axis',(-1.,7.99858039355471E-31,-1.4081690688991E-16));
#128980=DIRECTION('center_axis',(-1.4081690688991E-16,-6.98296267768627E-15,
1.));
#128981=DIRECTION('ref_axis',(-1.,7.99858039355471E-31,-1.4081690688991E-16));
#128982=DIRECTION('center_axis',(-1.4081690688991E-16,-6.98296267768627E-15,
1.));
#128983=DIRECTION('ref_axis',(-1.,7.99858039355471E-31,-1.4081690688991E-16));
#128984=DIRECTION('',(0.203374579494966,-0.456775406784111,-0.866022521746666));
#128985=DIRECTION('center_axis',(-1.4081690688991E-16,-6.98296267768627E-15,
1.));
#128986=DIRECTION('ref_axis',(-1.,9.83319205199467E-31,-1.40816906889911E-16));
#128987=DIRECTION('',(-0.500000000000004,0.866025403784436,5.97701461910994E-15));
#128988=DIRECTION('center_axis',(1.4081690688991E-16,6.98296267768627E-15,
-1.));
#128989=DIRECTION('ref_axis',(-1.,8.01265634860448E-31,-1.4081690688991E-16));
#128990=DIRECTION('',(0.406736643075804,-0.913545457642599,-6.32197843909137E-15));
#128991=DIRECTION('center_axis',(-1.4081690688991E-16,-6.98296267768627E-15,
1.));
#128992=DIRECTION('ref_axis',(-1.,8.32577322149061E-31,-1.39145123902276E-16));
#128993=DIRECTION('center_axis',(-0.866560035746415,-0.499072844768497,
-7.86457190912175E-6));
#128994=DIRECTION('ref_axis',(-7.54612232684255E-6,-2.65573230665248E-6,
0.999999999968002));
#128995=DIRECTION('center_axis',(0.913109622086441,0.407714137590671,-7.86457235765693E-6));
#128996=DIRECTION('ref_axis',(0.345763669669472,-0.774356189803008,0.529924500330442));
#128997=DIRECTION('center_axis',(-1.4081690688991E-16,-6.98296267768627E-15,
1.));
#128998=DIRECTION('ref_axis',(-1.,8.07722881720021E-31,-1.42096112075504E-16));
#128999=DIRECTION('center_axis',(-0.86653727315328,-0.499112366246934,9.77058997059964E-6));
#129000=DIRECTION('ref_axis',(0.436548602172256,-0.757907285851671,0.484769908301251));
#129001=DIRECTION('center_axis',(0.913128216134695,0.407672492085507,9.77051465153252E-6));
#129002=DIRECTION('ref_axis',(0.356566110901248,-0.798668832019048,0.48475633602676));
#129003=DIRECTION('center_axis',(-1.4081690688991E-16,-6.98296267768627E-15,
1.));
#129004=DIRECTION('ref_axis',(-1.,8.24049048117772E-31,-1.37719829560012E-16));
#129005=DIRECTION('center_axis',(0.864723324094334,0.502248516610423,-1.81624797431789E-5));
#129006=DIRECTION('ref_axis',(0.434560065157393,-0.748201970507551,-0.501349539841237));
#129007=DIRECTION('center_axis',(-0.914599195355563,-0.404361609857069,
-1.81316451872637E-5));
#129008=DIRECTION('ref_axis',(0.350582289842822,-0.792936907583349,-0.498340364249896));
#129009=DIRECTION('center_axis',(-1.4081690688991E-16,-6.98296267768627E-15,
1.));
#129010=DIRECTION('ref_axis',(-1.,8.26087817385229E-31,-1.38060560438432E-16));
#129011=DIRECTION('center_axis',(0.864716537642879,0.502260200677778,-1.84940595705526E-5));
#129012=DIRECTION('ref_axis',(0.435458542074697,-0.74968907742123,0.498339387696262));
#129013=DIRECTION('center_axis',(-0.914604658795487,-0.404349252214455,
-1.85257175418162E-5));
#129014=DIRECTION('ref_axis',(0.34985285273649,-0.791361267750787,0.501348506865241));
#129015=DIRECTION('center_axis',(-1.4081690688991E-16,-6.98296267768627E-15,
1.));
#129016=DIRECTION('ref_axis',(-1.,9.83319205199467E-31,-1.40816906889911E-16));
#129017=DIRECTION('center_axis',(-1.4081690688991E-16,-6.98296267768627E-15,
1.));
#129018=DIRECTION('ref_axis',(-1.,8.46073526001725E-31,-1.4081690688991E-16));
#129019=DIRECTION('',(-0.406736643075804,0.913545457642599,6.32197843909137E-15));
#129020=DIRECTION('center_axis',(-1.4081690688991E-16,-6.98296267768627E-15,
1.));
#129021=DIRECTION('ref_axis',(-1.,7.97077743482043E-31,-1.4081690688991E-16));
#129022=DIRECTION('center_axis',(-1.4081690688991E-16,-6.98296267768627E-15,
1.));
#129023=DIRECTION('ref_axis',(-1.,7.97077743482043E-31,-1.4081690688991E-16));
#129024=DIRECTION('center_axis',(-1.4081690688991E-16,-6.98296267768627E-15,
1.));
#129025=DIRECTION('ref_axis',(-1.,7.97077743482043E-31,-1.4081690688991E-16));
#129026=DIRECTION('',(0.309016994374951,-0.951056516295152,-6.59767734033507E-15));
#129027=DIRECTION('center_axis',(1.4081690688991E-16,6.98296267768627E-15,
-1.));
#129028=DIRECTION('ref_axis',(1.,-7.97077743482043E-31,1.4081690688991E-16));
#129029=DIRECTION('',(-0.203374797931581,0.456775527877827,-0.866022406579773));
#129030=DIRECTION('center_axis',(1.4081690688991E-16,6.98296267768627E-15,
-1.));
#129031=DIRECTION('ref_axis',(-1.,7.97577417048809E-31,-1.40816906889911E-16));
#129032=DIRECTION('',(0.154505557223423,-0.475534671805169,0.866022406579778));
#129033=DIRECTION('center_axis',(-1.4081690688991E-16,-6.98296267768627E-15,
1.));
#129034=DIRECTION('ref_axis',(-1.,9.83319205199467E-31,-1.40816906889911E-16));
#129035=DIRECTION('center_axis',(-1.4081690688991E-16,-6.98296267768627E-15,
1.));
#129036=DIRECTION('ref_axis',(-1.,7.98248735348668E-31,-1.4081690688991E-16));
#129037=DIRECTION('',(-0.406736643075804,0.913545457642599,6.32197843909137E-15));
#129038=DIRECTION('center_axis',(1.4081690688991E-16,6.98296267768627E-15,
-1.));
#129039=DIRECTION('ref_axis',(-1.,7.98707387273907E-31,-1.4081690688991E-16));
#129040=DIRECTION('',(0.309016994374951,-0.951056516295152,-6.59767734033507E-15));
#129041=DIRECTION('center_axis',(-1.4081690688991E-16,-6.98296267768627E-15,
1.));
#129042=DIRECTION('ref_axis',(-1.,7.99150043815584E-31,-1.4081690688991E-16));
#129043=DIRECTION('center_axis',(-1.4081690688991E-16,-6.98296267768627E-15,
1.));
#129044=DIRECTION('ref_axis',(1.,-7.99370576998456E-31,1.4081690688991E-16));
#129045=DIRECTION('',(-0.203366124261499,0.456779171296629,0.866022521746647));
#129046=DIRECTION('center_axis',(-1.4081690688991E-16,-6.98296267768627E-15,
1.));
#129047=DIRECTION('ref_axis',(-1.,7.99858039355471E-31,-1.4081690688991E-16));
#129048=DIRECTION('center_axis',(-1.4081690688991E-16,-6.98296267768627E-15,
1.));
#129049=DIRECTION('ref_axis',(-1.,7.99858039355471E-31,-1.4081690688991E-16));
#129050=DIRECTION('center_axis',(-1.4081690688991E-16,-6.98296267768627E-15,
1.));
#129051=DIRECTION('ref_axis',(-1.,7.99858039355471E-31,-1.4081690688991E-16));
#129052=DIRECTION('',(0.154514440939472,-0.475531575574881,-0.866022521746654));
#129053=DIRECTION('center_axis',(-1.4081690688991E-16,-6.98296267768627E-15,
1.));
#129054=DIRECTION('ref_axis',(-1.,9.83319205199467E-31,-1.40816906889911E-16));
#129055=DIRECTION('',(-0.406736643075804,0.913545457642599,6.32197843909137E-15));
#129056=DIRECTION('center_axis',(1.4081690688991E-16,6.98296267768627E-15,
-1.));
#129057=DIRECTION('ref_axis',(-1.,8.01265634860448E-31,-1.4081690688991E-16));
#129058=DIRECTION('',(0.309016994374951,-0.951056516295152,-6.59767734033507E-15));
#129059=DIRECTION('center_axis',(-1.4081690688991E-16,-6.98296267768627E-15,
1.));
#129060=DIRECTION('ref_axis',(-1.,8.32577322149061E-31,-1.39145123902276E-16));
#129061=DIRECTION('center_axis',(-0.913980246723226,-0.405758682640185,
-7.86457207997714E-6));
#129062=DIRECTION('ref_axis',(-7.78238363794176E-6,-1.85239945587372E-6,
0.999999999968002));
#129063=DIRECTION('center_axis',(0.950725244291261,0.310034691293523,-7.86457239813168E-6));
#129064=DIRECTION('ref_axis',(0.262927277567293,-0.806256330617357,0.529924500330459));
#129065=DIRECTION('center_axis',(-1.4081690688991E-16,-6.98296267768627E-15,
1.));
#129066=DIRECTION('ref_axis',(-1.,8.07722881720021E-31,-1.42096112075504E-16));
#129067=DIRECTION('center_axis',(-0.913961739946,-0.405800366953278,9.77059292800127E-6));
#129068=DIRECTION('ref_axis',(0.354934259362583,-0.799387144963777,0.484769908304337));
#129069=DIRECTION('center_axis',(0.950739383338137,0.309991330321278,9.77051800362196E-6));
#129070=DIRECTION('ref_axis',(0.271129178767072,-0.831564948217509,0.484756336025744));
#129071=DIRECTION('center_axis',(-1.4081690688991E-16,-6.98296267768627E-15,
1.));
#129072=DIRECTION('ref_axis',(-1.,8.24049048117772E-31,-1.37719829560012E-16));
#129073=DIRECTION('center_axis',(0.912485544867181,0.409108946466059,-1.81624797516694E-5));
#129074=DIRECTION('ref_axis',(0.353971097460658,-0.789527137635661,-0.501349539841553));
#129075=DIRECTION('center_axis',(-0.951856222950087,-0.306544826252928,
-1.81316451597188E-5));
#129076=DIRECTION('ref_axis',(0.265777286958649,-0.825238944241719,-0.498340364252901));
#129077=DIRECTION('center_axis',(-1.4081690688991E-16,-6.98296267768627E-15,
1.));
#129078=DIRECTION('ref_axis',(-1.,8.26087817385229E-31,-1.38060560438432E-16));
#129079=DIRECTION('center_axis',(0.912480016913784,0.409121275896266,-1.84940747170214E-5));
#129080=DIRECTION('ref_axis',(0.354709207427226,-0.791100014434018,0.49833938769562));
#129081=DIRECTION('center_axis',(-0.951860364736425,-0.306531965218374,
-1.85257114665936E-5));
#129082=DIRECTION('ref_axis',(0.265216544996837,-0.823595688993655,0.501348506860256));
#129083=DIRECTION('center_axis',(-1.4081690688991E-16,-6.98296267768627E-15,
1.));
#129084=DIRECTION('ref_axis',(-1.,9.83319205199467E-31,-1.40816906889911E-16));
#129085=DIRECTION('center_axis',(-1.4081690688991E-16,-6.98296267768627E-15,
1.));
#129086=DIRECTION('ref_axis',(-1.,8.46073526001725E-31,-1.4081690688991E-16));
#129087=DIRECTION('',(-0.309016994374951,0.951056516295152,6.59767734033507E-15));
#129088=DIRECTION('center_axis',(-1.4081690688991E-16,-6.98296267768627E-15,
1.));
#129089=DIRECTION('ref_axis',(-1.,7.97077743482043E-31,-1.4081690688991E-16));
#129090=DIRECTION('center_axis',(-1.4081690688991E-16,-6.98296267768627E-15,
1.));
#129091=DIRECTION('ref_axis',(-1.,7.97077743482043E-31,-1.4081690688991E-16));
#129092=DIRECTION('center_axis',(-1.4081690688991E-16,-6.98296267768627E-15,
1.));
#129093=DIRECTION('ref_axis',(-1.,7.97077743482043E-31,-1.4081690688991E-16));
#129094=DIRECTION('',(0.207911690817763,-0.978147600733805,-6.80109070798532E-15));
#129095=DIRECTION('center_axis',(1.4081690688991E-16,6.98296267768627E-15,
-1.));
#129096=DIRECTION('ref_axis',(1.,-7.97077743482043E-31,1.4081690688991E-16));
#129097=DIRECTION('',(-0.15451464552171,0.475531718838027,-0.86602240657979));
#129098=DIRECTION('center_axis',(1.4081690688991E-16,6.98296267768627E-15,
-1.));
#129099=DIRECTION('ref_axis',(-1.,7.97577417048809E-31,-1.40816906889911E-16));
#129100=DIRECTION('',(0.103952251140481,-0.489079871579877,0.866022406579782));
#129101=DIRECTION('center_axis',(-1.4081690688991E-16,-6.98296267768627E-15,
1.));
#129102=DIRECTION('ref_axis',(-1.,9.83319205199467E-31,-1.40816906889911E-16));
#129103=DIRECTION('center_axis',(-1.4081690688991E-16,-6.98296267768627E-15,
1.));
#129104=DIRECTION('ref_axis',(-1.,7.98248735348668E-31,-1.4081690688991E-16));
#129105=DIRECTION('',(-0.309016994374951,0.951056516295152,6.59767734033507E-15));
#129106=DIRECTION('center_axis',(1.4081690688991E-16,6.98296267768627E-15,
-1.));
#129107=DIRECTION('ref_axis',(-1.,7.98707387273907E-31,-1.4081690688991E-16));
#129108=DIRECTION('',(0.207911690817763,-0.978147600733805,-6.80109070798532E-15));
#129109=DIRECTION('center_axis',(-1.4081690688991E-16,-6.98296267768627E-15,
1.));
#129110=DIRECTION('ref_axis',(-1.,7.99150043815584E-31,-1.4081690688991E-16));
#129111=DIRECTION('center_axis',(-1.4081690688991E-16,-6.98296267768627E-15,
1.));
#129112=DIRECTION('ref_axis',(1.,-7.99370576998456E-31,1.4081690688991E-16));
#129113=DIRECTION('',(-0.15450563852595,0.475534435652397,0.86602252174666));
#129114=DIRECTION('center_axis',(-1.4081690688991E-16,-6.98296267768627E-15,
1.));
#129115=DIRECTION('ref_axis',(-1.,7.99858039355471E-31,-1.4081690688991E-16));
#129116=DIRECTION('center_axis',(-1.4081690688991E-16,-6.98296267768627E-15,
1.));
#129117=DIRECTION('ref_axis',(-1.,7.99858039355471E-31,-1.4081690688991E-16));
#129118=DIRECTION('center_axis',(-1.4081690688991E-16,-6.98296267768627E-15,
1.));
#129119=DIRECTION('ref_axis',(-1.,7.99858039355471E-31,-1.4081690688991E-16));
#129120=DIRECTION('',(0.103961409834821,-0.489077720912281,-0.866022521746637));
#129121=DIRECTION('center_axis',(-1.4081690688991E-16,-6.98296267768627E-15,
1.));
#129122=DIRECTION('ref_axis',(-1.,9.83319205199467E-31,-1.40816906889911E-16));
#129123=DIRECTION('',(-0.309016994374951,0.951056516295152,6.59767734033507E-15));
#129124=DIRECTION('center_axis',(1.4081690688991E-16,6.98296267768627E-15,
-1.));
#129125=DIRECTION('ref_axis',(-1.,8.01265634860448E-31,-1.4081690688991E-16));
#129126=DIRECTION('',(0.207911690817763,-0.978147600733805,-6.80109070798532E-15));
#129127=DIRECTION('center_axis',(-1.4081690688991E-16,-6.98296267768627E-15,
1.));
#129128=DIRECTION('ref_axis',(-1.,8.32577322149061E-31,-1.39145123902276E-16));
#129129=DIRECTION('center_axis',(-0.95138669885423,-0.307998943474485,-7.8645720778757E-6));
#129130=DIRECTION('ref_axis',(-7.93337939628674E-6,-1.02877119897231E-6,
0.999999999968002));
#129131=DIRECTION('center_axis',(0.977924521767604,0.208958440039522,-7.86457220880847E-6));
#129132=DIRECTION('ref_axis',(0.177210199190816,-0.829322958353561,0.529924500330424));
#129133=DIRECTION('center_axis',(-1.4081690688991E-16,-6.98296267768627E-15,
1.));
#129134=DIRECTION('ref_axis',(-1.,8.07722881720021E-31,-1.42096112075504E-16));
#129135=DIRECTION('center_axis',(-0.951372650655529,-0.308042333923779,
9.77058867857651E-6));
#129136=DIRECTION('ref_axis',(0.269431182533647,-0.832108751235263,0.484769908303116));
#129137=DIRECTION('center_axis',(0.977934050903442,0.208913838670687,9.77051839951797E-6));
#129138=DIRECTION('ref_axis',(0.182721698612432,-0.855350264825644,0.484756336027584));
#129139=DIRECTION('center_axis',(-1.4081690688991E-16,-6.98296267768627E-15,
1.));
#129140=DIRECTION('ref_axis',(-1.,8.24049048117772E-31,-1.37719829560012E-16));
#129141=DIRECTION('center_axis',(0.950250383060611,0.311487093092615,-1.8162479738927E-5));
#129142=DIRECTION('ref_axis',(0.269503948346045,-0.82220208022195,-0.501349539846792));
#129143=DIRECTION('center_axis',(-0.978684514577287,-0.205369473383614,
-1.81316452205297E-5));
#129144=DIRECTION('ref_axis',(0.178060372501871,-0.848499490336936,-0.498340364251638));
#129145=DIRECTION('center_axis',(-1.4081690688991E-16,-6.98296267768627E-15,
1.));
#129146=DIRECTION('ref_axis',(-1.,8.26087817385229E-31,-1.38060560438432E-16));
#129147=DIRECTION('center_axis',(0.95024617416422,0.311499932815776,-1.84940629314651E-5));
#129148=DIRECTION('ref_axis',(0.270073604475813,-0.823843494141799,0.498339387692437));
#129149=DIRECTION('center_axis',(-0.97868728932903,-0.205356249874684,-1.85257221081351E-5));
#129150=DIRECTION('ref_axis',(0.177674469289125,-0.846806623517829,0.501348506858415));
#129151=DIRECTION('center_axis',(-1.4081690688991E-16,-6.98296267768627E-15,
1.));
#129152=DIRECTION('ref_axis',(-1.,9.83319205199467E-31,-1.40816906889911E-16));
#129153=DIRECTION('center_axis',(-1.4081690688991E-16,-6.98296267768627E-15,
1.));
#129154=DIRECTION('ref_axis',(-1.,8.46073526001725E-31,-1.4081690688991E-16));
#129155=DIRECTION('',(-0.207911690817763,0.978147600733805,6.80109070798532E-15));
#129156=DIRECTION('center_axis',(-1.4081690688991E-16,-6.98296267768627E-15,
1.));
#129157=DIRECTION('ref_axis',(-1.,7.97077743482043E-31,-1.4081690688991E-16));
#129158=DIRECTION('center_axis',(-1.4081690688991E-16,-6.98296267768627E-15,
1.));
#129159=DIRECTION('ref_axis',(-1.,7.97077743482043E-31,-1.4081690688991E-16));
#129160=DIRECTION('center_axis',(-1.4081690688991E-16,-6.98296267768627E-15,
1.));
#129161=DIRECTION('ref_axis',(-1.,7.97077743482043E-31,-1.4081690688991E-16));
#129162=DIRECTION('',(0.104528463267657,-0.994521895368273,-6.92998990261915E-15));
#129163=DIRECTION('center_axis',(1.4081690688991E-16,6.98296267768627E-15,
-1.));
#129164=DIRECTION('ref_axis',(1.,-7.97077743482043E-31,1.4081690688991E-16));
#129165=DIRECTION('',(-0.103961598321241,0.48907788477527,-0.866022406579784));
#129166=DIRECTION('center_axis',(1.4081690688991E-16,6.98296267768627E-15,
-1.));
#129167=DIRECTION('ref_axis',(-1.,7.97577417048809E-31,-1.40816906889911E-16));
#129168=DIRECTION('',(0.0522600224406469,-0.497266609935018,0.866022406579782));
#129169=DIRECTION('center_axis',(-1.4081690688991E-16,-6.98296267768627E-15,
1.));
#129170=DIRECTION('ref_axis',(-1.,9.83319205199467E-31,-1.40816906889911E-16));
#129171=DIRECTION('center_axis',(-1.4081690688991E-16,-6.98296267768627E-15,
1.));
#129172=DIRECTION('ref_axis',(-1.,7.98248735348668E-31,-1.4081690688991E-16));
#129173=DIRECTION('',(-0.207911690817763,0.978147600733805,6.80109070798532E-15));
#129174=DIRECTION('center_axis',(1.4081690688991E-16,6.98296267768627E-15,
-1.));
#129175=DIRECTION('ref_axis',(-1.,7.98707387273907E-31,-1.4081690688991E-16));
#129176=DIRECTION('',(0.104528463267657,-0.994521895368273,-6.92998990261915E-15));
#129177=DIRECTION('center_axis',(-1.4081690688991E-16,-6.98296267768627E-15,
1.));
#129178=DIRECTION('ref_axis',(-1.,7.99150043815584E-31,-1.4081690688991E-16));
#129179=DIRECTION('center_axis',(-1.4081690688991E-16,-6.98296267768627E-15,
1.));
#129180=DIRECTION('ref_axis',(1.,-7.99370576998456E-31,1.4081690688991E-16));
#129181=DIRECTION('',(-0.103952356682308,0.489079645219203,0.866022521746665));
#129182=DIRECTION('center_axis',(-1.4081690688991E-16,-6.98296267768627E-15,
1.));
#129183=DIRECTION('ref_axis',(-1.,7.99858039355471E-31,-1.4081690688991E-16));
#129184=DIRECTION('center_axis',(-1.4081690688991E-16,-6.98296267768627E-15,
1.));
#129185=DIRECTION('ref_axis',(-1.,7.99858039355471E-31,-1.4081690688991E-16));
#129186=DIRECTION('center_axis',(-1.4081690688991E-16,-6.98296267768627E-15,
1.));
#129187=DIRECTION('ref_axis',(-1.,7.99858039355471E-31,-1.4081690688991E-16));
#129188=DIRECTION('',(0.0522693557686684,-0.497265428393196,-0.866022521746669));
#129189=DIRECTION('center_axis',(-1.4081690688991E-16,-6.98296267768627E-15,
1.));
#129190=DIRECTION('ref_axis',(-1.,9.83319205199467E-31,-1.40816906889911E-16));
#129191=DIRECTION('',(-0.207911690817763,0.978147600733805,6.80109070798532E-15));
#129192=DIRECTION('center_axis',(1.4081690688991E-16,6.98296267768627E-15,
-1.));
#129193=DIRECTION('ref_axis',(-1.,8.01265634860448E-31,-1.4081690688991E-16));
#129194=DIRECTION('',(0.104528463267657,-0.994521895368273,-6.92998990261915E-15));
#129195=DIRECTION('center_axis',(-1.4081690688991E-16,-6.98296267768627E-15,
1.));
#129196=DIRECTION('ref_axis',(-1.,8.32577322149061E-31,-1.39145123902276E-16));
#129197=DIRECTION('center_axis',(-0.97836955922212,-0.206864703431162,-7.86457204713208E-6));
#129198=DIRECTION('ref_axis',(-7.99745536701625E-6,-1.93871482032999E-7,
0.999999999968002));
#129199=DIRECTION('center_axis',(0.994409453539566,0.1055927963892,-7.86457224402987E-6));
#129200=DIRECTION('ref_axis',(0.089551568788591,-0.843303350210964,0.52992450033044));
#129201=DIRECTION('center_axis',(-1.4081690688991E-16,-6.98296267768627E-15,
1.));
#129202=DIRECTION('ref_axis',(-1.,8.07722881720021E-31,-1.42096112075504E-16));
#129203=DIRECTION('center_axis',(-0.978360123517457,-0.206909324621784,
9.77058473225947E-6));
#129204=DIRECTION('ref_axis',(0.180976161286408,-0.855713599897275,0.484769908303809));
#129205=DIRECTION('center_axis',(0.994414268361371,0.10554744328432,9.77051646637645E-6));
#129206=DIRECTION('ref_axis',(0.0923122812912403,-0.869764184940697,0.484756336025897));
#129207=DIRECTION('center_axis',(-1.4081690688991E-16,-6.98296267768627E-15,
1.));
#129208=DIRECTION('ref_axis',(-1.,8.24049048117772E-31,-1.37719829560012E-16));
#129209=DIRECTION('center_axis',(0.977604079204538,0.21045252194443,-1.81624797767727E-5));
#129210=DIRECTION('ref_axis',(0.182084057577967,-0.845868804766416,-0.501349539841195));
#129211=DIRECTION('center_axis',(-0.994790133859859,-0.101944049587639,
-1.81316452111653E-5));
#129212=DIRECTION('ref_axis',(0.088392591342371,-0.862463698456793,-0.498340364249185));
#129213=DIRECTION('center_axis',(-1.4081690688991E-16,-6.98296267768627E-15,
1.));
#129214=DIRECTION('ref_axis',(-1.,8.26087817385229E-31,-1.38060560438432E-16));
#129215=DIRECTION('center_axis',(0.977601235480708,0.210465731283179,-1.84940567618171E-5));
#129216=DIRECTION('ref_axis',(0.182479018595484,-0.84756077212075,0.498339387701301));
#129217=DIRECTION('center_axis',(-0.994791511178781,-0.101930608471819,
-1.85257114470306E-5));
#129218=DIRECTION('ref_axis',(0.0881857549149666,-0.860739767469655,0.501348506855623));
#129219=DIRECTION('center_axis',(-1.4081690688991E-16,-6.98296267768627E-15,
1.));
#129220=DIRECTION('ref_axis',(-1.,9.83319205199467E-31,-1.40816906889911E-16));
#129221=DIRECTION('center_axis',(-1.4081690688991E-16,-6.98296267768627E-15,
1.));
#129222=DIRECTION('ref_axis',(-1.,8.46073526001725E-31,-1.4081690688991E-16));
#129223=DIRECTION('',(-0.104528463267657,0.994521895368273,6.92998990261915E-15));
#129224=DIRECTION('center_axis',(-1.4081690688991E-16,-6.98296267768627E-15,
1.));
#129225=DIRECTION('ref_axis',(-1.,7.97077743482043E-31,-1.4081690688991E-16));
#129226=DIRECTION('center_axis',(-1.4081690688991E-16,-6.98296267768627E-15,
1.));
#129227=DIRECTION('ref_axis',(-1.,7.97077743482043E-31,-1.4081690688991E-16));
#129228=DIRECTION('center_axis',(-1.4081690688991E-16,-6.98296267768627E-15,
1.));
#129229=DIRECTION('ref_axis',(-1.,7.97077743482043E-31,-1.4081690688991E-16));
#129230=DIRECTION('',(3.49148133884313E-15,-1.,-6.98296267768627E-15));
#129231=DIRECTION('center_axis',(1.4081690688991E-16,6.98296267768627E-15,
-1.));
#129232=DIRECTION('ref_axis',(1.,-7.97077743482043E-31,1.4081690688991E-16));
#129233=DIRECTION('',(-0.0522695260941984,0.497265611060783,-0.86602240657978));
#129234=DIRECTION('center_axis',(1.4081690688991E-16,6.98296267768627E-15,
-1.));
#129235=DIRECTION('ref_axis',(-1.,7.97577417048809E-31,-1.40816906889911E-16));
#129236=DIRECTION('',(-4.77800116381158E-6,-0.500005191251988,0.86602240657978));
#129237=DIRECTION('center_axis',(-1.4081690688991E-16,-6.98296267768627E-15,
1.));
#129238=DIRECTION('ref_axis',(-1.,9.83319205199467E-31,-1.40816906889911E-16));
#129239=DIRECTION('center_axis',(-1.4081690688991E-16,-6.98296267768627E-15,
1.));
#129240=DIRECTION('ref_axis',(-1.,7.98248735348668E-31,-1.4081690688991E-16));
#129241=DIRECTION('',(-0.104528463267657,0.994521895368273,6.92998990261915E-15));
#129242=DIRECTION('center_axis',(1.4081690688991E-16,6.98296267768627E-15,
-1.));
#129243=DIRECTION('ref_axis',(-1.,7.98707387273907E-31,-1.4081690688991E-16));
#129244=DIRECTION('',(3.49148133884313E-15,-1.,-6.98296267768627E-15));
#129245=DIRECTION('center_axis',(-1.4081690688991E-16,-6.98296267768627E-15,
1.));
#129246=DIRECTION('ref_axis',(-1.,7.99150043815584E-31,-1.4081690688991E-16));
#129247=DIRECTION('center_axis',(-1.4081690688991E-16,-6.98296267768627E-15,
1.));
#129248=DIRECTION('ref_axis',(1.,-7.99370576998456E-31,1.4081690688991E-16));
#129249=DIRECTION('',(-0.0522601510654385,0.497266395846527,0.866022521746648));
#129250=DIRECTION('center_axis',(-1.4081690688991E-16,-6.98296267768627E-15,
1.));
#129251=DIRECTION('ref_axis',(-1.,7.99858039355471E-31,-1.4081690688991E-16));
#129252=DIRECTION('center_axis',(-1.4081690688991E-16,-6.98296267768627E-15,
1.));
#129253=DIRECTION('ref_axis',(-1.,7.99858039355471E-31,-1.4081690688991E-16));
#129254=DIRECTION('center_axis',(-1.4081690688991E-16,-6.98296267768627E-15,
1.));
#129255=DIRECTION('ref_axis',(-1.,7.99858039355471E-31,-1.4081690688991E-16));
#129256=DIRECTION('',(4.62770265447403E-6,-0.500004991781227,-0.866022521746657));
#129257=DIRECTION('center_axis',(-1.4081690688991E-16,-6.98296267768627E-15,
1.));
#129258=DIRECTION('ref_axis',(-1.,9.83319205199467E-31,-1.40816906889911E-16));
#129259=DIRECTION('',(-0.104528463267657,0.994521895368273,6.92998990261915E-15));
#129260=DIRECTION('center_axis',(1.4081690688991E-16,6.98296267768627E-15,
-1.));
#129261=DIRECTION('ref_axis',(-1.,8.01265634860448E-31,-1.4081690688991E-16));
#129262=DIRECTION('',(3.49148133884313E-15,-1.,-6.98296267768627E-15));
#129263=DIRECTION('center_axis',(-1.4081690688991E-16,-6.98296267768627E-15,
1.));
#129264=DIRECTION('ref_axis',(-1.,8.32577322149061E-31,-1.39145123902276E-16));
#129265=DIRECTION('center_axis',(-0.994633197962183,-0.103464010407821,
-7.86457204165851E-6));
#129266=DIRECTION('ref_axis',(-7.97390954732109E-6,6.43152258466824E-7,
0.999999999968002));
#129267=DIRECTION('center_axis',(0.999999427244995,0.00107025596491169,
-7.8645722516888E-6));
#129268=DIRECTION('ref_axis',(0.000911792658824946,-0.848044334090887,0.529924500330464));
#129269=DIRECTION('center_axis',(-1.4081690688991E-16,-6.98296267768627E-15,
1.));
#129270=DIRECTION('ref_axis',(-1.,8.07722881720021E-31,-1.42096112075504E-16));
#129271=DIRECTION('center_axis',(-0.994628478131894,-0.103509373457524,
9.77058659696217E-6));
#129272=DIRECTION('ref_axis',(0.0905383273445894,-0.869943071290438,0.484769908302283));
#129273=DIRECTION('center_axis',(0.999999475000345,0.00102464802303793,
9.77051626642102E-6));
#129274=DIRECTION('ref_axis',(0.000891471298433148,-0.874648786634365,0.484756336026624));
#129275=DIRECTION('center_axis',(-1.4081690688991E-16,-6.98296267768627E-15,
1.));
#129276=DIRECTION('ref_axis',(-1.,8.24049048117772E-31,-1.37719829560012E-16));
#129277=DIRECTION('center_axis',(0.994246940479906,0.107112188925769,-1.81624797621619E-5));
#129278=DIRECTION('ref_axis',(0.0926692157700999,-0.860268013669517,-0.501349539847857));
#129279=DIRECTION('center_axis',(-0.999996624262643,0.00259829454877836,
-1.81316452333963E-5));
#129280=DIRECTION('ref_axis',(0.00224363754548965,0.866978573814012,0.498340364247155));
#129281=DIRECTION('center_axis',(-1.4081690688991E-16,-6.98296267768627E-15,
1.));
#129282=DIRECTION('ref_axis',(-1.,8.26087817385229E-31,-1.38060560438432E-16));
#129283=DIRECTION('center_axis',(0.994245493086127,0.107125623152885,-1.84940559963087E-5));
#129284=DIRECTION('ref_axis',(0.0928851544033258,-0.861991996926722,0.498339387692517));
#129285=DIRECTION('center_axis',(-0.999996589057286,0.00261180600205774,
-1.85257109659478E-5));
#129286=DIRECTION('ref_axis',(0.00226914104443498,0.865242466405694,-0.50134850685637));
#129287=DIRECTION('center_axis',(-1.4081690688991E-16,-6.98296267768627E-15,
1.));
#129288=DIRECTION('ref_axis',(-1.,9.83319205199467E-31,-1.40816906889911E-16));
#129289=DIRECTION('center_axis',(-1.4081690688991E-16,-6.98296267768627E-15,
1.));
#129290=DIRECTION('ref_axis',(-1.,8.46073526001725E-31,-1.4081690688991E-16));
#129291=DIRECTION('',(-3.49148133884313E-15,1.,6.98296267768627E-15));
#129292=DIRECTION('center_axis',(-1.4081690688991E-16,-6.98296267768627E-15,
1.));
#129293=DIRECTION('ref_axis',(-1.,7.97077743482043E-31,-1.4081690688991E-16));
#129294=DIRECTION('center_axis',(-1.4081690688991E-16,-6.98296267768627E-15,
1.));
#129295=DIRECTION('ref_axis',(-1.,7.97077743482043E-31,-1.4081690688991E-16));
#129296=DIRECTION('center_axis',(-1.4081690688991E-16,-6.98296267768627E-15,
1.));
#129297=DIRECTION('ref_axis',(-1.,7.97077743482043E-31,-1.4081690688991E-16));
#129298=DIRECTION('',(-0.10452846326765,-0.994521895368274,-6.95942865237777E-15));
#129299=DIRECTION('center_axis',(1.4081690688991E-16,6.98296267768627E-15,
-1.));
#129300=DIRECTION('ref_axis',(1.,-7.97077743482043E-31,1.4081690688991E-16));
#129301=DIRECTION('',(-4.77800116722347E-6,0.500005191251988,-0.86602240657978));
#129302=DIRECTION('center_axis',(1.4081690688991E-16,6.98296267768627E-15,
-1.));
#129303=DIRECTION('ref_axis',(-1.,7.97577417048809E-31,-1.40816906889911E-16));
#129304=DIRECTION('',(-0.0522695260941984,-0.497265611060783,0.86602240657978));
#129305=DIRECTION('center_axis',(-1.4081690688991E-16,-6.98296267768627E-15,
1.));
#129306=DIRECTION('ref_axis',(-1.,9.83319205199467E-31,-1.40816906889911E-16));
#129307=DIRECTION('center_axis',(-1.4081690688991E-16,-6.98296267768627E-15,
1.));
#129308=DIRECTION('ref_axis',(-1.,7.98248735348668E-31,-1.4081690688991E-16));
#129309=DIRECTION('',(-3.49148133884313E-15,1.,6.98296267768627E-15));
#129310=DIRECTION('center_axis',(1.4081690688991E-16,6.98296267768627E-15,
-1.));
#129311=DIRECTION('ref_axis',(-1.,7.98707387273907E-31,-1.4081690688991E-16));
#129312=DIRECTION('',(-0.10452846326765,-0.994521895368274,-6.95942865237777E-15));
#129313=DIRECTION('center_axis',(-1.4081690688991E-16,-6.98296267768627E-15,
1.));
#129314=DIRECTION('ref_axis',(-1.,7.99150043815584E-31,-1.4081690688991E-16));
#129315=DIRECTION('center_axis',(-1.4081690688991E-16,-6.98296267768627E-15,
1.));
#129316=DIRECTION('ref_axis',(1.,-7.99370576998456E-31,1.4081690688991E-16));
#129317=DIRECTION('',(4.62770265084889E-6,0.500004991781227,0.866022521746657));
#129318=DIRECTION('center_axis',(-1.4081690688991E-16,-6.98296267768627E-15,
1.));
#129319=DIRECTION('ref_axis',(-1.,7.99858039355471E-31,-1.4081690688991E-16));
#129320=DIRECTION('center_axis',(-1.4081690688991E-16,-6.98296267768627E-15,
1.));
#129321=DIRECTION('ref_axis',(-1.,7.99858039355471E-31,-1.4081690688991E-16));
#129322=DIRECTION('center_axis',(-1.4081690688991E-16,-6.98296267768627E-15,
1.));
#129323=DIRECTION('ref_axis',(-1.,7.99858039355471E-31,-1.4081690688991E-16));
#129324=DIRECTION('',(-0.0522601510654325,-0.497266395846506,-0.86602252174666));
#129325=DIRECTION('center_axis',(-1.4081690688991E-16,-6.98296267768627E-15,
1.));
#129326=DIRECTION('ref_axis',(-1.,9.83319205199467E-31,-1.40816906889911E-16));
#129327=DIRECTION('',(-3.49148133884313E-15,1.,6.98296267768627E-15));
#129328=DIRECTION('center_axis',(1.4081690688991E-16,6.98296267768627E-15,
-1.));
#129329=DIRECTION('ref_axis',(-1.,8.01265634860448E-31,-1.4081690688991E-16));
#129330=DIRECTION('',(-0.10452846326765,-0.994521895368274,-6.95942865237777E-15));
#129331=DIRECTION('center_axis',(-1.4081690688991E-16,-6.98296267768627E-15,
1.));
#129332=DIRECTION('ref_axis',(-1.,8.32577322149061E-31,-1.39145123902276E-16));
#129333=DIRECTION('center_axis',(-0.999999427244995,0.00107025596477908,
-7.86457202530775E-6));
#129334=DIRECTION('ref_axis',(-7.86299990295341E-6,1.47312954961576E-6,
0.999999999968002));
#129335=DIRECTION('center_axis',(0.994633197962195,-0.103464010407701,-7.86457224889578E-6));
#129336=DIRECTION('ref_axis',(-0.0877379732621264,-0.843493966781859,0.529924500330433));
#129337=DIRECTION('center_axis',(-1.4081690688991E-16,-6.98296267768627E-15,
1.));
#129338=DIRECTION('ref_axis',(-1.,8.07722881720021E-31,-1.42096112075504E-16));
#129339=DIRECTION('center_axis',(-0.999999475000305,0.00102464806168852,
9.7705860071373E-6));
#129340=DIRECTION('ref_axis',(0.000891463458118558,0.874641264344406,-0.484769908305911));
#129341=DIRECTION('center_axis',(0.994628478127856,-0.10350937349633,9.77051619636314E-6));
#129342=DIRECTION('ref_axis',(0.0905391058404323,0.869950553190108,-0.484756336026502));
#129343=DIRECTION('center_axis',(-1.4081690688991E-16,-6.98296267768627E-15,
1.));
#129344=DIRECTION('ref_axis',(-1.,8.24049048117772E-31,-1.37719829560012E-16));
#129345=DIRECTION('center_axis',(0.999996624215829,0.00259831235056682,
-1.81624797792608E-5));
#129346=DIRECTION('ref_axis',(0.00223907064277466,-0.865241946198171,-0.501349539844066));
#129347=DIRECTION('center_axis',(-0.994246942387264,0.107112171226335,-1.81316451412819E-5));
#129348=DIRECTION('ref_axis',(0.0928552846708738,0.861994650487102,0.498340364249486));
#129349=DIRECTION('center_axis',(-1.4081690688991E-16,-6.98296267768627E-15,
1.));
#129350=DIRECTION('ref_axis',(-1.,8.26087817385229E-31,-1.38060560438432E-16));
#129351=DIRECTION('center_axis',(0.999996589010146,0.00261182427508522,
-1.84940600871693E-5));
#129352=DIRECTION('ref_axis',(0.00227362102100115,-0.866979057022949,0.498339387697832));
#129353=DIRECTION('center_axis',(-0.994245495043239,0.10712560498323,-1.85257097907709E-5));
#129354=DIRECTION('ref_axis',(0.092699175819317,0.860265387813317,-0.501348506862066));
#129355=DIRECTION('center_axis',(-1.4081690688991E-16,-6.98296267768627E-15,
1.));
#129356=DIRECTION('ref_axis',(-1.,9.83319205199467E-31,-1.40816906889911E-16));
#129357=DIRECTION('center_axis',(-1.4081690688991E-16,-6.98296267768627E-15,
1.));
#129358=DIRECTION('ref_axis',(-1.,8.46073526001725E-31,-1.4081690688991E-16));
#129359=DIRECTION('',(0.10452846326765,0.994521895368274,6.95942865237777E-15));
#129360=DIRECTION('center_axis',(-1.4081690688991E-16,-6.98296267768627E-15,
1.));
#129361=DIRECTION('ref_axis',(-1.,7.97077743482043E-31,-1.4081690688991E-16));
#129362=DIRECTION('center_axis',(-1.4081690688991E-16,-6.98296267768627E-15,
1.));
#129363=DIRECTION('ref_axis',(-1.,7.97077743482043E-31,-1.4081690688991E-16));
#129364=DIRECTION('center_axis',(-1.4081690688991E-16,-6.98296267768627E-15,
1.));
#129365=DIRECTION('ref_axis',(-1.,7.97077743482043E-31,-1.4081690688991E-16));
#129366=DIRECTION('',(-0.207911690817756,-0.978147600733806,-6.85964567039975E-15));
#129367=DIRECTION('center_axis',(1.4081690688991E-16,6.98296267768627E-15,
-1.));
#129368=DIRECTION('ref_axis',(1.,-7.97077743482043E-31,1.4081690688991E-16));
#129369=DIRECTION('',(0.0522600224406469,0.497266609935018,-0.866022406579782));
#129370=DIRECTION('center_axis',(1.4081690688991E-16,6.98296267768627E-15,
-1.));
#129371=DIRECTION('ref_axis',(-1.,7.97577417048809E-31,-1.40816906889911E-16));
#129372=DIRECTION('',(-0.103961598321246,-0.48907788477529,0.866022406579772));
#129373=DIRECTION('center_axis',(-1.4081690688991E-16,-6.98296267768627E-15,
1.));
#129374=DIRECTION('ref_axis',(-1.,9.83319205199467E-31,-1.40816906889911E-16));
#129375=DIRECTION('center_axis',(-1.4081690688991E-16,-6.98296267768627E-15,
1.));
#129376=DIRECTION('ref_axis',(-1.,7.98248735348668E-31,-1.4081690688991E-16));
#129377=DIRECTION('',(0.10452846326765,0.994521895368274,6.95942865237777E-15));
#129378=DIRECTION('center_axis',(1.4081690688991E-16,6.98296267768627E-15,
-1.));
#129379=DIRECTION('ref_axis',(-1.,7.98707387273907E-31,-1.4081690688991E-16));
#129380=DIRECTION('',(-0.207911690817756,-0.978147600733806,-6.85964567039975E-15));
#129381=DIRECTION('center_axis',(-1.4081690688991E-16,-6.98296267768627E-15,
1.));
#129382=DIRECTION('ref_axis',(-1.,7.99150043815584E-31,-1.4081690688991E-16));
#129383=DIRECTION('center_axis',(-1.4081690688991E-16,-6.98296267768627E-15,
1.));
#129384=DIRECTION('ref_axis',(1.,-7.99370576998456E-31,1.4081690688991E-16));
#129385=DIRECTION('',(0.0522693557686642,0.497265428393217,0.866022521746657));
#129386=DIRECTION('center_axis',(-1.4081690688991E-16,-6.98296267768627E-15,
1.));
#129387=DIRECTION('ref_axis',(-1.,7.99858039355471E-31,-1.4081690688991E-16));
#129388=DIRECTION('center_axis',(-1.4081690688991E-16,-6.98296267768627E-15,
1.));
#129389=DIRECTION('ref_axis',(-1.,7.99858039355471E-31,-1.4081690688991E-16));
#129390=DIRECTION('center_axis',(-1.4081690688991E-16,-6.98296267768627E-15,
1.));
#129391=DIRECTION('ref_axis',(-1.,7.99858039355471E-31,-1.4081690688991E-16));
#129392=DIRECTION('',(-0.103952356682315,-0.489079645219203,-0.866022521746664));
#129393=DIRECTION('center_axis',(-1.4081690688991E-16,-6.98296267768627E-15,
1.));
#129394=DIRECTION('ref_axis',(-1.,9.83319205199467E-31,-1.40816906889911E-16));
#129395=DIRECTION('',(0.10452846326765,0.994521895368274,6.95942865237777E-15));
#129396=DIRECTION('center_axis',(1.4081690688991E-16,6.98296267768627E-15,
-1.));
#129397=DIRECTION('ref_axis',(-1.,8.01265634860448E-31,-1.4081690688991E-16));
#129398=DIRECTION('',(-0.207911690817756,-0.978147600733806,-6.85964567039975E-15));
#129399=DIRECTION('center_axis',(-1.4081690688991E-16,-6.98296267768627E-15,
1.));
#129400=DIRECTION('ref_axis',(-1.,8.32577322149061E-31,-1.39145123902276E-16));
#129401=DIRECTION('center_axis',(-0.99440945353958,0.105592796389069,-7.8645720232461E-6));
#129402=DIRECTION('ref_axis',(-7.66594160056427E-6,2.28696684648491E-6,
0.999999999968002));
#129403=DIRECTION('center_axis',(0.978369559222141,-0.206864703431062,-7.86457222351689E-6));
#129404=DIRECTION('ref_axis',(-0.175426463587687,-0.829702103060253,0.529924500330482));
#129405=DIRECTION('center_axis',(-1.4081690688991E-16,-6.98296267768627E-15,
1.));
#129406=DIRECTION('ref_axis',(-1.,8.07722881720021E-31,-1.42096112075504E-16));
#129407=DIRECTION('center_axis',(-0.994414268357388,0.105547443321838,9.77058454997984E-6));
#129408=DIRECTION('ref_axis',(0.0923114872006156,0.869756704679602,-0.484769908302578));
#129409=DIRECTION('center_axis',(0.97836012350987,-0.206909324657662,9.77051847768451E-6));
#129410=DIRECTION('ref_axis',(0.180977717589303,0.855720959436757,-0.484756336025433));
#129411=DIRECTION('center_axis',(-1.4081690688991E-16,-6.98296267768627E-15,
1.));
#129412=DIRECTION('ref_axis',(-1.,8.24049048117772E-31,-1.37719829560012E-16));
#129413=DIRECTION('center_axis',(0.994790135674088,-0.101944031878547,-1.81624797219411E-5));
#129414=DIRECTION('ref_axis',(0.0882156062118037,0.860736106903253,0.501349539835948));
#129415=DIRECTION('center_axis',(-0.977604082951534,0.210452504541368,-1.81316451866862E-5));
#129416=DIRECTION('ref_axis',(0.18244958986568,0.847566533384385,0.498340364253811));
#129417=DIRECTION('center_axis',(-1.4081690688991E-16,-6.98296267768627E-15,
1.));
#129418=DIRECTION('ref_axis',(-1.,8.26087817385229E-31,-1.38060560438432E-16));
#129419=DIRECTION('center_axis',(0.994791513041809,-0.101930590295349,-1.84940629635532E-5));
#129420=DIRECTION('ref_axis',(0.0883628226288196,0.862467313147628,-0.498339387695754));
#129421=DIRECTION('center_axis',(-0.977601239326386,0.210465713417443,-1.85257108287527E-5));
#129422=DIRECTION('ref_axis',(0.182113579025484,0.845863061613818,-0.501348506861073));
#129423=DIRECTION('center_axis',(-1.4081690688991E-16,-6.98296267768627E-15,
1.));
#129424=DIRECTION('ref_axis',(-1.,9.83319205199467E-31,-1.40816906889911E-16));
#129425=DIRECTION('center_axis',(-1.4081690688991E-16,-6.98296267768627E-15,
1.));
#129426=DIRECTION('ref_axis',(-1.,8.46073526001725E-31,-1.4081690688991E-16));
#129427=DIRECTION('',(0.207911690817756,0.978147600733806,6.85964567039975E-15));
#129428=DIRECTION('center_axis',(-1.4081690688991E-16,-6.98296267768627E-15,
1.));
#129429=DIRECTION('ref_axis',(-1.,7.97077743482043E-31,-1.4081690688991E-16));
#129430=DIRECTION('center_axis',(-1.4081690688991E-16,-6.98296267768627E-15,
1.));
#129431=DIRECTION('ref_axis',(-1.,7.97077743482043E-31,-1.4081690688991E-16));
#129432=DIRECTION('center_axis',(-1.4081690688991E-16,-6.98296267768627E-15,
1.));
#129433=DIRECTION('ref_axis',(-1.,7.97077743482043E-31,-1.4081690688991E-16));
#129434=DIRECTION('',(-0.309016994374945,-0.951056516295154,-6.68470697498368E-15));
#129435=DIRECTION('center_axis',(1.4081690688991E-16,6.98296267768627E-15,
-1.));
#129436=DIRECTION('ref_axis',(1.,-7.97077743482043E-31,1.4081690688991E-16));
#129437=DIRECTION('',(0.103952251140481,0.489079871579877,-0.866022406579782));
#129438=DIRECTION('center_axis',(1.4081690688991E-16,6.98296267768627E-15,
-1.));
#129439=DIRECTION('ref_axis',(-1.,7.97577417048809E-31,-1.40816906889911E-16));
#129440=DIRECTION('',(-0.154514645521688,-0.47553171883805,0.866022406579782));
#129441=DIRECTION('center_axis',(-1.4081690688991E-16,-6.98296267768627E-15,
1.));
#129442=DIRECTION('ref_axis',(-1.,9.83319205199467E-31,-1.40816906889911E-16));
#129443=DIRECTION('center_axis',(-1.4081690688991E-16,-6.98296267768627E-15,
1.));
#129444=DIRECTION('ref_axis',(-1.,7.98248735348668E-31,-1.4081690688991E-16));
#129445=DIRECTION('',(0.207911690817756,0.978147600733806,6.85964567039975E-15));
#129446=DIRECTION('center_axis',(1.4081690688991E-16,6.98296267768627E-15,
-1.));
#129447=DIRECTION('ref_axis',(-1.,7.98707387273907E-31,-1.4081690688991E-16));
#129448=DIRECTION('',(-0.309016994374945,-0.951056516295154,-6.68470697498368E-15));
#129449=DIRECTION('center_axis',(-1.4081690688991E-16,-6.98296267768627E-15,
1.));
#129450=DIRECTION('ref_axis',(-1.,7.99150043815584E-31,-1.4081690688991E-16));
#129451=DIRECTION('center_axis',(-1.4081690688991E-16,-6.98296267768627E-15,
1.));
#129452=DIRECTION('ref_axis',(1.,-7.99370576998456E-31,1.4081690688991E-16));
#129453=DIRECTION('',(0.103961409834803,0.489077720912241,0.866022521746662));
#129454=DIRECTION('center_axis',(-1.4081690688991E-16,-6.98296267768627E-15,
1.));
#129455=DIRECTION('ref_axis',(-1.,7.99858039355471E-31,-1.4081690688991E-16));
#129456=DIRECTION('center_axis',(-1.4081690688991E-16,-6.98296267768627E-15,
1.));
#129457=DIRECTION('ref_axis',(-1.,7.99858039355471E-31,-1.4081690688991E-16));
#129458=DIRECTION('center_axis',(-1.4081690688991E-16,-6.98296267768627E-15,
1.));
#129459=DIRECTION('ref_axis',(-1.,7.99858039355471E-31,-1.4081690688991E-16));
#129460=DIRECTION('',(-0.154505638525963,-0.475534435652396,-0.866022521746659));
#129461=DIRECTION('center_axis',(-1.4081690688991E-16,-6.98296267768627E-15,
1.));
#129462=DIRECTION('ref_axis',(-1.,9.83319205199467E-31,-1.40816906889911E-16));
#129463=DIRECTION('',(0.207911690817756,0.978147600733806,6.85964567039975E-15));
#129464=DIRECTION('center_axis',(1.4081690688991E-16,6.98296267768627E-15,
-1.));
#129465=DIRECTION('ref_axis',(-1.,8.01265634860448E-31,-1.4081690688991E-16));
#129466=DIRECTION('',(-0.309016994374945,-0.951056516295154,-6.68470697498368E-15));
#129467=DIRECTION('center_axis',(-1.4081690688991E-16,-6.98296267768627E-15,
1.));
#129468=DIRECTION('ref_axis',(-1.,8.32577322149061E-31,-1.39145123902276E-16));
#129469=DIRECTION('center_axis',(-0.977924521767628,0.208958440039413,-7.86457201262958E-6));
#129470=DIRECTION('ref_axis',(-7.38489362573486E-6,3.07574770634862E-6,
0.999999999968002));
#129471=DIRECTION('center_axis',(0.951386698854285,-0.307998943474316,-7.86457238851017E-6));
#129472=DIRECTION('ref_axis',(-0.26119294486766,-0.806819849471295,0.529924500330449));
#129473=DIRECTION('center_axis',(-1.4081690688991E-16,-6.98296267768627E-15,
1.));
#129474=DIRECTION('ref_axis',(-1.,8.07722881720021E-31,-1.42096112075504E-16));
#129475=DIRECTION('center_axis',(-0.977934050895432,0.208913838708178,9.77058768185539E-6));
#129476=DIRECTION('ref_axis',(0.182720126971878,0.855342908548244,-0.484769908302497));
#129477=DIRECTION('center_axis',(0.951372650643604,-0.308042333960611,9.77051871801589E-6));
#129478=DIRECTION('ref_axis',(0.269433499591928,0.832115907779339,-0.484756336026888));
#129479=DIRECTION('center_axis',(-1.4081690688991E-16,-6.98296267768627E-15,
1.));
#129480=DIRECTION('ref_axis',(-1.,8.24049048117772E-31,-1.37719829560012E-16));
#129481=DIRECTION('center_axis',(0.978684518232685,-0.205369455961155,-1.81624797422718E-5));
#129482=DIRECTION('ref_axis',(0.177703774423219,0.846799862690149,0.50134953984589));
#129483=DIRECTION('center_axis',(-0.950250388606176,0.311487076176613,-1.81316452346279E-5));
#129484=DIRECTION('ref_axis',(0.270044939174658,0.82385229998126,0.498340364250924));
#129485=DIRECTION('center_axis',(-1.4081690688991E-16,-6.98296267768627E-15,
1.));
#129486=DIRECTION('ref_axis',(-1.,8.26087817385229E-31,-1.38060560438432E-16));
#129487=DIRECTION('center_axis',(0.978687293082038,-0.205356231991439,-1.84940717020688E-5));
#129488=DIRECTION('ref_axis',(0.178031144703119,0.848506196906769,-0.498339387693276));
#129489=DIRECTION('center_axis',(-0.950246179854334,0.311499915455917,-1.85257060786387E-5));
#129490=DIRECTION('ref_axis',(0.269532707750638,0.822193282704124,-0.50134850685808));
#129491=DIRECTION('center_axis',(-1.4081690688991E-16,-6.98296267768627E-15,
1.));
#129492=DIRECTION('ref_axis',(-1.,9.83319205199467E-31,-1.40816906889911E-16));
#129493=DIRECTION('center_axis',(-1.4081690688991E-16,-6.98296267768627E-15,
1.));
#129494=DIRECTION('ref_axis',(-1.,8.46073526001725E-31,-1.4081690688991E-16));
#129495=DIRECTION('',(0.309016994374945,0.951056516295154,6.68470697498368E-15));
#129496=DIRECTION('center_axis',(-1.4081690688991E-16,-6.98296267768627E-15,
1.));
#129497=DIRECTION('ref_axis',(-1.,7.97077743482043E-31,-1.4081690688991E-16));
#129498=DIRECTION('center_axis',(-1.4081690688991E-16,-6.98296267768627E-15,
1.));
#129499=DIRECTION('ref_axis',(-1.,7.97077743482043E-31,-1.4081690688991E-16));
#129500=DIRECTION('center_axis',(-1.4081690688991E-16,-6.98296267768627E-15,
1.));
#129501=DIRECTION('ref_axis',(-1.,7.97077743482043E-31,-1.4081690688991E-16));
#129502=DIRECTION('',(-0.406736643075798,-0.913545457642602,-6.43652923108483E-15));
#129503=DIRECTION('center_axis',(1.4081690688991E-16,6.98296267768627E-15,
-1.));
#129504=DIRECTION('ref_axis',(1.,-7.97077743482043E-31,1.4081690688991E-16));
#129505=DIRECTION('',(0.154505557223428,0.47553467180519,-0.866022406579765));
#129506=DIRECTION('center_axis',(1.4081690688991E-16,6.98296267768627E-15,
-1.));
#129507=DIRECTION('ref_axis',(-1.,7.97577417048809E-31,-1.40816906889911E-16));
#129508=DIRECTION('',(-0.203374797931581,-0.456775527877827,0.866022406579773));
#129509=DIRECTION('center_axis',(-1.4081690688991E-16,-6.98296267768627E-15,
1.));
#129510=DIRECTION('ref_axis',(-1.,9.83319205199467E-31,-1.40816906889911E-16));
#129511=DIRECTION('center_axis',(-1.4081690688991E-16,-6.98296267768627E-15,
1.));
#129512=DIRECTION('ref_axis',(-1.,7.98248735348668E-31,-1.4081690688991E-16));
#129513=DIRECTION('',(0.309016994374945,0.951056516295154,6.68470697498368E-15));
#129514=DIRECTION('center_axis',(1.4081690688991E-16,6.98296267768627E-15,
-1.));
#129515=DIRECTION('ref_axis',(-1.,7.98707387273907E-31,-1.4081690688991E-16));
#129516=DIRECTION('',(-0.406736643075798,-0.913545457642602,-6.43652923108483E-15));
#129517=DIRECTION('center_axis',(-1.4081690688991E-16,-6.98296267768627E-15,
1.));
#129518=DIRECTION('ref_axis',(-1.,7.99150043815584E-31,-1.4081690688991E-16));
#129519=DIRECTION('center_axis',(-1.4081690688991E-16,-6.98296267768627E-15,
1.));
#129520=DIRECTION('ref_axis',(1.,-7.99370576998456E-31,1.4081690688991E-16));
#129521=DIRECTION('',(0.154514440939479,0.47553157557488,0.866022521746653));
#129522=DIRECTION('center_axis',(-1.4081690688991E-16,-6.98296267768627E-15,
1.));
#129523=DIRECTION('ref_axis',(-1.,7.99858039355471E-31,-1.4081690688991E-16));
#129524=DIRECTION('center_axis',(-1.4081690688991E-16,-6.98296267768627E-15,
1.));
#129525=DIRECTION('ref_axis',(-1.,7.99858039355471E-31,-1.4081690688991E-16));
#129526=DIRECTION('center_axis',(-1.4081690688991E-16,-6.98296267768627E-15,
1.));
#129527=DIRECTION('ref_axis',(-1.,7.99858039355471E-31,-1.4081690688991E-16));
#129528=DIRECTION('',(-0.203366124261494,-0.456779171296591,-0.866022521746668));
#129529=DIRECTION('center_axis',(-1.4081690688991E-16,-6.98296267768627E-15,
1.));
#129530=DIRECTION('ref_axis',(-1.,9.83319205199467E-31,-1.40816906889911E-16));
#129531=DIRECTION('',(0.309016994374945,0.951056516295154,6.68470697498368E-15));
#129532=DIRECTION('center_axis',(1.4081690688991E-16,6.98296267768627E-15,
-1.));
#129533=DIRECTION('ref_axis',(-1.,8.01265634860448E-31,-1.4081690688991E-16));
#129534=DIRECTION('',(-0.406736643075798,-0.913545457642602,-6.43652923108483E-15));
#129535=DIRECTION('center_axis',(-1.4081690688991E-16,-6.98296267768627E-15,
1.));
#129536=DIRECTION('ref_axis',(-1.,8.32577322149061E-31,-1.39145123902276E-16));
#129537=DIRECTION('center_axis',(-0.950725244291359,0.310034691293224,-7.86457185161666E-6));
#129538=DIRECTION('ref_axis',(-7.02293506467738E-6,3.83082999767987E-6,
0.999999999968002));
#129539=DIRECTION('center_axis',(0.913980246723279,-0.405758682640066,-7.86457228997838E-6));
#129540=DIRECTION('ref_axis',(-0.344097741585765,-0.775097908773538,0.529924500330438));
#129541=DIRECTION('center_axis',(-1.4081690688991E-16,-6.98296267768627E-15,
1.));
#129542=DIRECTION('ref_axis',(-1.,8.07722881720021E-31,-1.42096112075504E-16));
#129543=DIRECTION('center_axis',(-0.950739383327522,0.309991330353832,9.77057983430093E-6));
#129544=DIRECTION('ref_axis',(0.271126846795281,0.83155779651818,-0.484769908303596));
#129545=DIRECTION('center_axis',(0.913961739929012,-0.405800366991542,9.77051730791796E-6));
#129546=DIRECTION('ref_axis',(0.354937311790441,0.799394020105231,-0.484756336027671));
#129547=DIRECTION('center_axis',(-1.4081690688991E-16,-6.98296267768627E-15,
1.));
#129548=DIRECTION('ref_axis',(-1.,8.24049048117772E-31,-1.37719829560012E-16));
#129549=DIRECTION('center_axis',(0.951856228406634,-0.30654480930791,-1.81624798152503E-5));
#129550=DIRECTION('ref_axis',(0.265244982896449,0.823585901985077,0.501349539841905));
#129551=DIRECTION('center_axis',(-0.912485552150597,0.409108930222335,-1.8131645163321E-5));
#129552=DIRECTION('ref_axis',(0.354681619617918,0.791111768373005,0.498340364256145));
#129553=DIRECTION('center_axis',(-1.4081690688991E-16,-6.98296267768627E-15,
1.));
#129554=DIRECTION('ref_axis',(-1.,8.26087817385229E-31,-1.38060560438432E-16));
#129555=DIRECTION('center_axis',(0.951860370339,-0.306531947822854,-1.84940563905878E-5));
#129556=DIRECTION('ref_axis',(0.265748920300046,0.825248669208596,-0.498339387695576));
#129557=DIRECTION('center_axis',(-0.912480024380723,0.409121259241015,-1.85256897665016E-5));
#129558=DIRECTION('ref_axis',(0.353998779726462,0.78951538213359,-0.501348506855887));
#129559=DIRECTION('center_axis',(-1.4081690688991E-16,-6.98296267768627E-15,
1.));
#129560=DIRECTION('ref_axis',(-1.,9.83319205199467E-31,-1.40816906889911E-16));
#129561=DIRECTION('center_axis',(-1.4081690688991E-16,-6.98296267768627E-15,
1.));
#129562=DIRECTION('ref_axis',(-1.,8.46073526001725E-31,-1.4081690688991E-16));
#129563=DIRECTION('',(0.406736643075798,0.913545457642602,6.43652923108483E-15));
#129564=DIRECTION('center_axis',(-1.4081690688991E-16,-6.98296267768627E-15,
1.));
#129565=DIRECTION('ref_axis',(-1.,7.97077743482043E-31,-1.4081690688991E-16));
#129566=DIRECTION('center_axis',(-1.4081690688991E-16,-6.98296267768627E-15,
1.));
#129567=DIRECTION('ref_axis',(-1.,7.97077743482043E-31,-1.4081690688991E-16));
#129568=DIRECTION('center_axis',(-1.4081690688991E-16,-6.98296267768627E-15,
1.));
#129569=DIRECTION('ref_axis',(-1.,7.97077743482043E-31,-1.4081690688991E-16));
#129570=DIRECTION('',(-0.499999999999998,-0.86602540378444,-6.11783152599987E-15));
#129571=DIRECTION('center_axis',(1.4081690688991E-16,6.98296267768627E-15,
-1.));
#129572=DIRECTION('ref_axis',(1.,-7.97077743482043E-31,1.4081690688991E-16));
#129573=DIRECTION('',(0.203366068089045,0.456779414654155,-0.866022406579766));
#129574=DIRECTION('center_axis',(1.4081690688991E-16,6.98296267768627E-15,
-1.));
#129575=DIRECTION('ref_axis',(-1.,-5.32907051820075E-15,-1.40816906889948E-16));
#129576=DIRECTION('',(-0.250006733496381,-0.433014808647736,0.86602240657978));
#129577=DIRECTION('center_axis',(-1.4081690688991E-16,-6.98296267768627E-15,
1.));
#129578=DIRECTION('ref_axis',(-1.,9.83319205199467E-31,-1.40816906889911E-16));
#129579=DIRECTION('center_axis',(-1.4081690688991E-16,-6.98296267768627E-15,
1.));
#129580=DIRECTION('ref_axis',(-1.,7.98248735348668E-31,-1.4081690688991E-16));
#129581=DIRECTION('',(0.406736643075798,0.913545457642602,6.43652923108483E-15));
#129582=DIRECTION('center_axis',(1.4081690688991E-16,6.98296267768627E-15,
-1.));
#129583=DIRECTION('ref_axis',(-1.,4.44089209850063E-15,-1.40816906889879E-16));
#129584=DIRECTION('',(-0.499999999999998,-0.86602540378444,-6.11783152599987E-15));
#129585=DIRECTION('center_axis',(-1.4081690688991E-16,-6.98296267768627E-15,
1.));
#129586=DIRECTION('ref_axis',(-1.,7.99150043815584E-31,-1.4081690688991E-16));
#129587=DIRECTION('center_axis',(-1.4081690688991E-16,-6.98296267768627E-15,
1.));
#129588=DIRECTION('ref_axis',(1.,-7.99370576998456E-31,1.4081690688991E-16));
#129589=DIRECTION('',(0.203374579494977,0.456775406784131,0.866022521746654));
#129590=DIRECTION('center_axis',(-1.4081690688991E-16,-6.98296267768627E-15,
1.));
#129591=DIRECTION('ref_axis',(-1.,7.99858039355471E-31,-1.4081690688991E-16));
#129592=DIRECTION('center_axis',(-1.4081690688991E-16,-6.98296267768627E-15,
1.));
#129593=DIRECTION('ref_axis',(-1.,7.99858039355471E-31,-1.4081690688991E-16));
#129594=DIRECTION('center_axis',(-1.4081690688991E-16,-6.98296267768627E-15,
1.));
#129595=DIRECTION('ref_axis',(-1.,7.99858039355471E-31,-1.4081690688991E-16));
#129596=DIRECTION('',(-0.249998488182568,-0.433019338752903,-0.866022521746651));
#129597=DIRECTION('center_axis',(-1.4081690688991E-16,-6.98296267768627E-15,
1.));
#129598=DIRECTION('ref_axis',(-1.,9.83319205199467E-31,-1.40816906889911E-16));
#129599=DIRECTION('',(0.406736643075798,0.913545457642602,6.43652923108483E-15));
#129600=DIRECTION('center_axis',(1.4081690688991E-16,6.98296267768627E-15,
-1.));
#129601=DIRECTION('ref_axis',(-1.,4.44089209850063E-15,-1.40816906889879E-16));
#129602=DIRECTION('',(-0.499999999999998,-0.86602540378444,-6.11783152599987E-15));
#129603=DIRECTION('center_axis',(-1.4081690688991E-16,-6.98296267768627E-15,
1.));
#129604=DIRECTION('ref_axis',(-1.,8.32577322149061E-31,-1.39145123902276E-16));
#129605=DIRECTION('center_axis',(-0.9131096220865,0.40771413759054,-7.8645720700241E-6));
#129606=DIRECTION('ref_axis',(-6.5840321423447E-6,4.54394095516308E-6,0.999999999968002));
#129607=DIRECTION('center_axis',(0.866560035746487,-0.499072844768372,-7.86457221102025E-6));
#129608=DIRECTION('ref_axis',(-0.423232531439977,-0.734883833187562,0.529924500330438));
#129609=DIRECTION('center_axis',(-1.4081690688991E-16,-6.98296267768627E-15,
1.));
#129610=DIRECTION('ref_axis',(-1.,8.07722881720021E-31,-1.42096112075504E-16));
#129611=DIRECTION('center_axis',(-0.913128216116196,0.407672492126938,9.77059649425398E-6));
#129612=DIRECTION('ref_axis',(0.356563044148269,0.798661963255189,-0.484769908304018));
#129613=DIRECTION('center_axis',(0.866537273133727,-0.499112366280882,9.77051914612337E-6));
#129614=DIRECTION('ref_axis',(0.436552356525903,0.757913804263692,-0.484756336026894));
#129615=DIRECTION('center_axis',(-1.4081690688991E-16,-6.98296267768627E-15,
1.));
#129616=DIRECTION('ref_axis',(-1.,8.24049048117772E-31,-1.37719829560012E-16));
#129617=DIRECTION('center_axis',(0.91459920255343,-0.404361593575297,-1.81624797483359E-5));
#129618=DIRECTION('ref_axis',(0.349880111830071,0.791348561788269,0.501349539843626));
#129619=DIRECTION('center_axis',(-0.864723333035792,0.502248501216991,-1.81316450871321E-5));
#129620=DIRECTION('ref_axis',(0.435432334017441,0.749703650685568,0.498340364250033));
#129621=DIRECTION('center_axis',(-1.4081690688991E-16,-6.98296267768627E-15,
1.));
#129622=DIRECTION('ref_axis',(-1.,8.26087817385229E-31,-1.38060560438432E-16));
#129623=DIRECTION('center_axis',(0.914604666183639,-0.404349235504512,-1.84940712939604E-5));
#129624=DIRECTION('ref_axis',(0.350555095115197,0.792949544397979,-0.498339387694583));
#129625=DIRECTION('center_axis',(-0.864716546823295,0.502260184871142,-1.85257210458366E-5));
#129626=DIRECTION('ref_axis',(0.434586366990142,0.748187385814829,-0.501348506863122));
#129627=DIRECTION('center_axis',(-1.4081690688991E-16,-6.98296267768627E-15,
1.));
#129628=DIRECTION('ref_axis',(-1.,9.83319205199467E-31,-1.40816906889911E-16));
#129629=DIRECTION('center_axis',(-1.4081690688991E-16,-6.98296267768627E-15,
1.));
#129630=DIRECTION('ref_axis',(-1.,8.46073526001725E-31,-1.4081690688991E-16));
#129631=DIRECTION('',(0.499999999999998,0.86602540378444,6.11783152599987E-15));
#129632=DIRECTION('center_axis',(-1.4081690688991E-16,-6.98296267768627E-15,
1.));
#129633=DIRECTION('ref_axis',(-1.,7.97077743482043E-31,-1.4081690688991E-16));
#129634=DIRECTION('center_axis',(-1.4081690688991E-16,-6.98296267768627E-15,
1.));
#129635=DIRECTION('ref_axis',(-1.,7.97077743482043E-31,-1.4081690688991E-16));
#129636=DIRECTION('center_axis',(-1.4081690688991E-16,-6.98296267768627E-15,
1.));
#129637=DIRECTION('ref_axis',(-1.,7.97077743482043E-31,-1.4081690688991E-16));
#129638=DIRECTION('',(-0.587785252292471,-0.809016994374949,-5.73210557847752E-15));
#129639=DIRECTION('center_axis',(1.4081690688991E-16,6.98296267768627E-15,
-1.));
#129640=DIRECTION('ref_axis',(1.,-7.97077743482043E-31,1.4081690688991E-16));
#129641=DIRECTION('',(0.24999845775561,0.433019586648882,-0.866022406579788));
#129642=DIRECTION('center_axis',(1.4081690688991E-16,6.98296267768627E-15,
-1.));
#129643=DIRECTION('ref_axis',(-1.,7.97577417048809E-31,-1.40816906889911E-16));
#129644=DIRECTION('',(-0.293899542971744,-0.404509888559955,0.866022406579768));
#129645=DIRECTION('center_axis',(-1.4081690688991E-16,-6.98296267768627E-15,
1.));
#129646=DIRECTION('ref_axis',(-1.,9.83319205199467E-31,-1.40816906889911E-16));
#129647=DIRECTION('center_axis',(-1.4081690688991E-16,-6.98296267768627E-15,
1.));
#129648=DIRECTION('ref_axis',(-1.,7.98248735348668E-31,-1.4081690688991E-16));
#129649=DIRECTION('',(0.499999999999998,0.86602540378444,6.11783152599987E-15));
#129650=DIRECTION('center_axis',(1.4081690688991E-16,6.98296267768627E-15,
-1.));
#129651=DIRECTION('ref_axis',(-1.,7.98707387273907E-31,-1.4081690688991E-16));
#129652=DIRECTION('',(-0.587785252292471,-0.809016994374949,-5.73210557847752E-15));
#129653=DIRECTION('center_axis',(-1.4081690688991E-16,-6.98296267768627E-15,
1.));
#129654=DIRECTION('ref_axis',(-1.,7.99150043815584E-31,-1.4081690688991E-16));
#129655=DIRECTION('center_axis',(-1.4081690688991E-16,-6.98296267768627E-15,
1.));
#129656=DIRECTION('ref_axis',(1.,-7.99370576998456E-31,1.4081690688991E-16));
#129657=DIRECTION('',(0.250006503598672,0.433014711050232,0.866022521746664));
#129658=DIRECTION('center_axis',(-1.4081690688991E-16,-6.98296267768627E-15,
1.));
#129659=DIRECTION('ref_axis',(-1.,7.99858039355471E-31,-1.4081690688991E-16));
#129660=DIRECTION('center_axis',(-1.4081690688991E-16,-6.98296267768627E-15,
1.));
#129661=DIRECTION('ref_axis',(-1.,7.99858039355471E-31,-1.4081690688991E-16));
#129662=DIRECTION('center_axis',(-1.4081690688991E-16,-6.98296267768627E-15,
1.));
#129663=DIRECTION('ref_axis',(-1.,7.99858039355471E-31,-1.4081690688991E-16));
#129664=DIRECTION('',(-0.293891816351551,-0.404515255718677,-0.866022521746657));
#129665=DIRECTION('center_axis',(-1.4081690688991E-16,-6.98296267768627E-15,
1.));
#129666=DIRECTION('ref_axis',(-1.,9.83319205199467E-31,-1.40816906889911E-16));
#129667=DIRECTION('',(0.499999999999998,0.86602540378444,6.11783152599987E-15));
#129668=DIRECTION('center_axis',(1.4081690688991E-16,6.98296267768627E-15,
-1.));
#129669=DIRECTION('ref_axis',(-1.,8.01265634860448E-31,-1.4081690688991E-16));
#129670=DIRECTION('',(-0.587785252292471,-0.809016994374949,-5.73210557847752E-15));
#129671=DIRECTION('center_axis',(-1.4081690688991E-16,-6.98296267768627E-15,
1.));
#129672=DIRECTION('ref_axis',(-1.,8.32577322149061E-31,-1.39145123902276E-16));
#129673=DIRECTION('center_axis',(-0.865489779781644,0.500926582476584,-7.86457211702301E-6));
#129674=DIRECTION('ref_axis',(-6.07299298703037E-6,5.20726757706905E-6,
0.999999999968002));
#129675=DIRECTION('center_axis',(0.809645611678812,-0.586919060371522,-7.86457243086484E-6));
#129676=DIRECTION('ref_axis',(-0.497730297112349,-0.686618216541007,0.529924500330471));
#129677=DIRECTION('center_axis',(-1.4081690688991E-16,-6.98296267768627E-15,
1.));
#129678=DIRECTION('ref_axis',(-1.,8.07722881720021E-31,-1.42096112075504E-16));
#129679=DIRECTION('center_axis',(-0.865512625090032,0.50088710875236,9.7705877695898E-6));
#129680=DIRECTION('ref_axis',(0.438092662174206,0.757015822392589,-0.484769908303299));
#129681=DIRECTION('center_axis',(0.809618842641174,-0.586955986037201,9.7705258656919E-6));
#129682=DIRECTION('ref_axis',(0.513384442288674,0.708129726178612,-0.484756336026824));
#129683=DIRECTION('center_axis',(-1.4081690688991E-16,-6.98296267768627E-15,
1.));
#129684=DIRECTION('ref_axis',(-1.,8.24049048117772E-31,-1.37719829560012E-16));
#129685=DIRECTION('center_axis',(0.867321636444868,-0.497748107605364,-1.81624797230982E-5));
#129686=DIRECTION('ref_axis',(0.430681881041376,0.750441041148587,0.501349539844694));
#129687=DIRECTION('center_axis',(-0.807487024129147,0.589885332530228,-1.81316452770967E-5));
#129688=DIRECTION('ref_axis',(0.511412360643298,0.700081622911464,0.498340364252085));
#129689=DIRECTION('center_axis',(-1.4081690688991E-16,-6.98296267768627E-15,
1.));
#129690=DIRECTION('ref_axis',(-1.,8.26087817385229E-31,-1.38060560438432E-16));
#129691=DIRECTION('center_axis',(0.867328361917146,-0.497736388334316,-1.84940634502467E-5));
#129692=DIRECTION('ref_axis',(0.431520514948145,0.751962698440445,-0.498339387699841));
#129693=DIRECTION('center_axis',(-0.807479053808288,0.589896242840782,-1.85256928077167E-5));
#129694=DIRECTION('ref_axis',(0.510412535077489,0.69866209193516,-0.501348506857811));
#129695=DIRECTION('center_axis',(-1.4081690688991E-16,-6.98296267768627E-15,
1.));
#129696=DIRECTION('ref_axis',(-1.,9.83319205199467E-31,-1.40816906889911E-16));
#129697=DIRECTION('center_axis',(-1.4081690688991E-16,-6.98296267768627E-15,
1.));
#129698=DIRECTION('ref_axis',(-1.,8.46073526001725E-31,-1.4081690688991E-16));
#129699=DIRECTION('',(0.587785252292471,0.809016994374949,5.73210557847752E-15));
#129700=DIRECTION('center_axis',(-1.4081690688991E-16,-6.98296267768627E-15,
1.));
#129701=DIRECTION('ref_axis',(-1.,7.97077743482043E-31,-1.4081690688991E-16));
#129702=DIRECTION('center_axis',(-1.4081690688991E-16,-6.98296267768627E-15,
1.));
#129703=DIRECTION('ref_axis',(-1.,7.97077743482043E-31,-1.4081690688991E-16));
#129704=DIRECTION('center_axis',(-1.4081690688991E-16,-6.98296267768627E-15,
1.));
#129705=DIRECTION('ref_axis',(-1.,7.97077743482043E-31,-1.4081690688991E-16));
#129706=DIRECTION('',(-0.669130606358857,-0.743144825477395,-5.28357748271715E-15));
#129707=DIRECTION('center_axis',(1.4081690688991E-16,6.98296267768627E-15,
-1.));
#129708=DIRECTION('ref_axis',(1.,-7.97077743482043E-31,1.4081690688991E-16));
#129709=DIRECTION('',(0.293891812003452,0.404515505437167,-0.866022406579784));
#129710=DIRECTION('center_axis',(1.4081690688991E-16,6.98296267768627E-15,
-1.));
#129711=DIRECTION('ref_axis',(-1.,7.97577417048809E-31,-1.40816906889911E-16));
#129712=DIRECTION('',(-0.334572327551836,-0.371573073483925,0.866022406579793));
#129713=DIRECTION('center_axis',(-1.4081690688991E-16,-6.98296267768627E-15,
1.));
#129714=DIRECTION('ref_axis',(-1.,9.83319205199467E-31,-1.40816906889911E-16));
#129715=DIRECTION('center_axis',(-1.4081690688991E-16,-6.98296267768627E-15,
1.));
#129716=DIRECTION('ref_axis',(-1.,7.98248735348668E-31,-1.4081690688991E-16));
#129717=DIRECTION('',(0.587785252292471,0.809016994374949,5.73210557847752E-15));
#129718=DIRECTION('center_axis',(1.4081690688991E-16,6.98296267768627E-15,
-1.));
#129719=DIRECTION('ref_axis',(-1.,7.98707387273907E-31,-1.4081690688991E-16));
#129720=DIRECTION('',(-0.669130606358857,-0.743144825477395,-5.28357748271715E-15));
#129721=DIRECTION('center_axis',(-1.4081690688991E-16,-6.98296267768627E-15,
1.));
#129722=DIRECTION('ref_axis',(-1.,7.99150043815584E-31,-1.4081690688991E-16));
#129723=DIRECTION('center_axis',(-1.4081690688991E-16,-6.98296267768627E-15,
1.));
#129724=DIRECTION('ref_axis',(1.,-7.99370576998456E-31,1.4081690688991E-16));
#129725=DIRECTION('',(0.293899304131716,0.404509815527969,0.866022521746647));
#129726=DIRECTION('center_axis',(-1.4081690688991E-16,-6.98296267768627E-15,
1.));
#129727=DIRECTION('ref_axis',(-1.,7.99858039355471E-31,-1.4081690688991E-16));
#129728=DIRECTION('center_axis',(-1.4081690688991E-16,-6.98296267768627E-15,
1.));
#129729=DIRECTION('ref_axis',(-1.,7.99858039355471E-31,-1.4081690688991E-16));
#129730=DIRECTION('center_axis',(-1.4081690688991E-16,-6.98296267768627E-15,
1.));
#129731=DIRECTION('ref_axis',(-1.,7.99858039355471E-31,-1.4081690688991E-16));
#129732=DIRECTION('',(-0.334565204279747,-0.371579218892574,-0.866022521746655));
#129733=DIRECTION('center_axis',(-1.4081690688991E-16,-6.98296267768627E-15,
1.));
#129734=DIRECTION('ref_axis',(-1.,9.83319205199467E-31,-1.40816906889911E-16));
#129735=DIRECTION('',(0.587785252292471,0.809016994374949,5.73210557847752E-15));
#129736=DIRECTION('center_axis',(1.4081690688991E-16,6.98296267768627E-15,
-1.));
#129737=DIRECTION('ref_axis',(-1.,8.01265634860448E-31,-1.4081690688991E-16));
#129738=DIRECTION('',(-0.669130606358857,-0.743144825477395,-5.28357748271715E-15));
#129739=DIRECTION('center_axis',(-1.4081690688991E-16,-6.98296267768627E-15,
1.));
#129740=DIRECTION('ref_axis',(-1.,8.32577322149061E-31,-1.39145123902276E-16));
#129741=DIRECTION('center_axis',(-0.808387450334232,0.588650770899239,-7.86457176580283E-6));
#129742=DIRECTION('ref_axis',(-5.49541651871241E-6,5.81354205727288E-6,
0.999999999968002));
#129743=DIRECTION('center_axis',(0.743860540860255,-0.668334867928674,-7.8645722585724E-6));
#129744=DIRECTION('ref_axis',(-0.566774825493092,-0.630829867029758,0.529924500330465));
#129745=DIRECTION('center_axis',(-1.4081690688991E-16,-6.98296267768627E-15,
1.));
#129746=DIRECTION('ref_axis',(-1.,8.07722881720021E-31,-1.42096112075504E-16));
#129747=DIRECTION('center_axis',(-0.808414296620484,0.588613901402391,9.77059021400816E-6));
#129748=DIRECTION('ref_axis',(0.514822445316503,0.70707565776395,-0.484769908302912));
#129749=DIRECTION('center_axis',(0.74383005867795,-0.668368793191075,9.77051183441469E-6));
#129750=DIRECTION('ref_axis',(0.584591780669533,0.650587230628282,-0.484756336025686));
#129751=DIRECTION('center_axis',(-1.4081690688991E-16,-6.98296267768627E-15,
1.));
#129752=DIRECTION('ref_axis',(-1.,8.24049048117772E-31,-1.37719829560012E-16));
#129753=DIRECTION('center_axis',(0.810541512988639,-0.585681189208098,-1.81624797439544E-5));
#129754=DIRECTION('ref_axis',(0.50676500943756,0.701311531421608,0.501349539847031));
#129755=DIRECTION('center_axis',(-0.741403718408824,0.671059256698552,-1.81316450741316E-5));
#129756=DIRECTION('ref_axis',(0.581789246426899,0.642789354376716,0.498340364251167));
#129757=DIRECTION('center_axis',(-1.4081690688991E-16,-6.98296267768627E-15,
1.));
#129758=DIRECTION('ref_axis',(-1.,8.26087817385229E-31,-1.38060560438432E-16));
#129759=DIRECTION('center_axis',(0.810549426613657,-0.585670237142235,-1.84940689245547E-5));
#129760=DIRECTION('ref_axis',(0.507758105718737,0.702737191802679,-0.498339387700997));
#129761=DIRECTION('center_axis',(-0.741394651315224,0.671069274112574,-1.85257009851561E-5));
#129762=DIRECTION('ref_axis',(0.580646516616596,0.641482109967114,-0.501348506862394));
#129763=DIRECTION('center_axis',(-1.4081690688991E-16,-6.98296267768627E-15,
1.));
#129764=DIRECTION('ref_axis',(-1.,9.83319205199467E-31,-1.40816906889911E-16));
#129765=DIRECTION('center_axis',(-1.4081690688991E-16,-6.98296267768627E-15,
1.));
#129766=DIRECTION('ref_axis',(-1.,8.46073526001725E-31,-1.4081690688991E-16));
#129767=DIRECTION('',(0.669130606358857,0.743144825477395,5.28357748271715E-15));
#129768=DIRECTION('center_axis',(-1.4081690688991E-16,-6.98296267768627E-15,
1.));
#129769=DIRECTION('ref_axis',(-1.,7.97077743482043E-31,-1.4081690688991E-16));
#129770=DIRECTION('center_axis',(-1.4081690688991E-16,-6.98296267768627E-15,
1.));
#129771=DIRECTION('ref_axis',(-1.,7.97077743482043E-31,-1.4081690688991E-16));
#129772=DIRECTION('center_axis',(-1.4081690688991E-16,-6.98296267768627E-15,
1.));
#129773=DIRECTION('ref_axis',(-1.,7.97077743482043E-31,-1.4081690688991E-16));
#129774=DIRECTION('',(-0.743144825477393,-0.669130606358859,-4.77716140639646E-15));
#129775=DIRECTION('center_axis',(1.4081690688991E-16,6.98296267768627E-15,
-1.));
#129776=DIRECTION('ref_axis',(1.,-7.97077743482043E-31,1.4081690688991E-16));
#129777=DIRECTION('',(0.334565226058181,0.371579467697516,-0.8660224065798));
#129778=DIRECTION('center_axis',(1.4081690688991E-16,6.98296267768627E-15,
-1.));
#129779=DIRECTION('ref_axis',(-1.,7.97577417048809E-31,-1.40816906889911E-16));
#129780=DIRECTION('',(-0.371579467697537,-0.334565226058201,0.866022406579784));
#129781=DIRECTION('center_axis',(-1.4081690688991E-16,-6.98296267768627E-15,
1.));
#129782=DIRECTION('ref_axis',(-1.,9.83319205199467E-31,-1.40816906889911E-16));
#129783=DIRECTION('center_axis',(-1.4081690688991E-16,-6.98296267768627E-15,
1.));
#129784=DIRECTION('ref_axis',(-1.,7.98248735348668E-31,-1.4081690688991E-16));
#129785=DIRECTION('',(0.669130606358857,0.743144825477395,5.28357748271715E-15));
#129786=DIRECTION('center_axis',(1.4081690688991E-16,6.98296267768627E-15,
-1.));
#129787=DIRECTION('ref_axis',(-1.,7.98707387273907E-31,-1.4081690688991E-16));
#129788=DIRECTION('',(-0.743144825477393,-0.669130606358859,-4.77716140639646E-15));
#129789=DIRECTION('center_axis',(-1.4081690688991E-16,-6.98296267768627E-15,
1.));
#129790=DIRECTION('ref_axis',(-1.,7.99150043815584E-31,-1.4081690688991E-16));
#129791=DIRECTION('center_axis',(-1.4081690688991E-16,-6.98296267768627E-15,
1.));
#129792=DIRECTION('ref_axis',(1.,8.88178419700124E-16,1.40816906889917E-16));
#129793=DIRECTION('',(0.334572082386297,0.3715730258176,0.866022521746663));
#129794=DIRECTION('center_axis',(-1.4081690688991E-16,-6.98296267768627E-15,
1.));
#129795=DIRECTION('ref_axis',(-1.,7.99858039355471E-31,-1.4081690688991E-16));
#129796=DIRECTION('center_axis',(-1.4081690688991E-16,-6.98296267768627E-15,
1.));
#129797=DIRECTION('ref_axis',(-1.,7.99858039355471E-31,-1.4081690688991E-16));
#129798=DIRECTION('center_axis',(-1.4081690688991E-16,-6.98296267768627E-15,
1.));
#129799=DIRECTION('ref_axis',(-1.,7.99858039355471E-31,-1.4081690688991E-16));
#129800=DIRECTION('',(-0.371573025817624,-0.334572082386294,-0.866022521746654));
#129801=DIRECTION('center_axis',(-1.4081690688991E-16,-6.98296267768627E-15,
1.));
#129802=DIRECTION('ref_axis',(-1.,9.83319205199467E-31,-1.40816906889911E-16));
#129803=DIRECTION('',(0.669130606358857,0.743144825477395,5.28357748271715E-15));
#129804=DIRECTION('center_axis',(1.4081690688991E-16,6.98296267768627E-15,
-1.));
#129805=DIRECTION('ref_axis',(-1.,1.06581410364015E-14,-1.40816906889836E-16));
#129806=DIRECTION('',(-0.743144825477393,-0.669130606358859,-4.77716140639646E-15));
#129807=DIRECTION('center_axis',(-1.4081690688991E-16,-6.98296267768627E-15,
1.));
#129808=DIRECTION('ref_axis',(-1.,8.32577322149061E-31,-1.39145123902276E-16));
#129809=DIRECTION('center_axis',(-0.742428258814693,0.66992557829324,-7.8645722868831E-6));
#129810=DIRECTION('ref_axis',(-4.85763186827067E-6,6.35612260159829E-6,
0.999999999968001));
#129811=DIRECTION('center_axis',(0.669925578293297,-0.742428258814641,-7.8645724034394E-6));
#129812=DIRECTION('ref_axis',(-0.629609650280272,-0.568130013485873,0.529924500330467));
#129813=DIRECTION('center_axis',(-1.4081690688991E-16,-6.98296267768627E-15,
1.));
#129814=DIRECTION('ref_axis',(-1.,8.07722881720021E-31,-1.42096112075504E-16));
#129815=DIRECTION('center_axis',(-0.742458811943861,0.669891716974801,9.77059652327666E-6));
#129816=DIRECTION('ref_axis',(0.585911726014692,0.649388624263867,-0.484769908302039));
#129817=DIRECTION('center_axis',(0.669891716946153,-0.742458811969709,9.77052689495564E-6));
#129818=DIRECTION('ref_axis',(0.649394209166457,0.585916765233755,-0.484756336027786));
#129819=DIRECTION('center_axis',(-1.4081690688991E-16,-6.98296267768627E-15,
1.));
#129820=DIRECTION('ref_axis',(-1.,8.24049048117772E-31,-1.37719829560012E-16));
#129821=DIRECTION('center_axis',(0.744880927099454,-0.667197425140102,-1.81624797771564E-5));
#129822=DIRECTION('ref_axis',(0.577295914345283,0.644498305800666,0.501349539842528));
#129823=DIRECTION('center_axis',(-0.667197438400621,0.744880915222623,-1.81316453516109E-5));
#129824=DIRECTION('ref_axis',(0.64579192747986,0.578454551163167,0.498340364249643));
#129825=DIRECTION('center_axis',(-1.4081690688991E-16,-6.98296267768627E-15,
1.));
#129826=DIRECTION('ref_axis',(-1.,8.26087817385229E-31,-1.38060560438432E-16));
#129827=DIRECTION('center_axis',(0.744889942174867,-0.667187360270481,-1.84940703591896E-5));
#129828=DIRECTION('ref_axis',(0.578432592428572,0.645812349435392,-0.498339387699889));
#129829=DIRECTION('center_axis',(-0.667187373871816,0.744889929991558,-1.85256986638901E-5));
#129830=DIRECTION('ref_axis',(0.644518813413593,0.57727391576619,-0.501348506861149));
#129831=DIRECTION('center_axis',(-1.4081690688991E-16,-6.98296267768627E-15,
1.));
#129832=DIRECTION('ref_axis',(-1.,9.83319205199467E-31,-1.40816906889911E-16));
#129833=DIRECTION('center_axis',(-1.4081690688991E-16,-6.98296267768627E-15,
1.));
#129834=DIRECTION('ref_axis',(-1.,8.46073526001725E-31,-1.4081690688991E-16));
#129835=DIRECTION('',(0.743144825477393,0.669130606358859,4.77716140639646E-15));
#129836=DIRECTION('center_axis',(-1.4081690688991E-16,-6.98296267768627E-15,
1.));
#129837=DIRECTION('ref_axis',(-1.,7.97077743482043E-31,-1.4081690688991E-16));
#129838=DIRECTION('center_axis',(-1.4081690688991E-16,-6.98296267768627E-15,
1.));
#129839=DIRECTION('ref_axis',(-1.,7.97077743482043E-31,-1.4081690688991E-16));
#129840=DIRECTION('center_axis',(-1.4081690688991E-16,-6.98296267768627E-15,
1.));
#129841=DIRECTION('ref_axis',(-1.,7.97077743482043E-31,-1.4081690688991E-16));
#129842=DIRECTION('',(-0.809016994374947,-0.587785252292474,-4.21840575002201E-15));
#129843=DIRECTION('center_axis',(1.4081690688991E-16,6.98296267768627E-15,
-1.));
#129844=DIRECTION('ref_axis',(1.,-7.97077743482043E-31,1.4081690688991E-16));
#129845=DIRECTION('',(0.3715730734839,0.334572327551839,-0.866022406579802));
#129846=DIRECTION('center_axis',(1.4081690688991E-16,6.98296267768627E-15,
-1.));
#129847=DIRECTION('ref_axis',(-1.,7.97577417048809E-31,-1.40816906889911E-16));
#129848=DIRECTION('',(-0.40451550543717,-0.293891812003427,0.866022406579791));
#129849=DIRECTION('center_axis',(-1.4081690688991E-16,-6.98296267768627E-15,
1.));
#129850=DIRECTION('ref_axis',(-1.,9.83319205199467E-31,-1.40816906889911E-16));
#129851=DIRECTION('center_axis',(-1.4081690688991E-16,-6.98296267768627E-15,
1.));
#129852=DIRECTION('ref_axis',(-1.,7.98248735348668E-31,-1.4081690688991E-16));
#129853=DIRECTION('',(0.743144825477393,0.669130606358859,4.77716140639646E-15));
#129854=DIRECTION('center_axis',(1.4081690688991E-16,6.98296267768627E-15,
-1.));
#129855=DIRECTION('ref_axis',(-1.,7.98707387273907E-31,-1.4081690688991E-16));
#129856=DIRECTION('',(-0.809016994374947,-0.587785252292474,-4.21840575002201E-15));
#129857=DIRECTION('center_axis',(-1.4081690688991E-16,-6.98296267768627E-15,
1.));
#129858=DIRECTION('ref_axis',(-1.,7.99150043815584E-31,-1.4081690688991E-16));
#129859=DIRECTION('center_axis',(-1.4081690688991E-16,-6.98296267768627E-15,
1.));
#129860=DIRECTION('ref_axis',(1.,-7.99370576998456E-31,1.4081690688991E-16));
#129861=DIRECTION('',(0.37157921889255,0.33456520427975,0.866022521746664));
#129862=DIRECTION('center_axis',(-1.4081690688991E-16,-6.98296267768627E-15,
1.));
#129863=DIRECTION('ref_axis',(-1.,7.99858039355471E-31,-1.4081690688991E-16));
#129864=DIRECTION('center_axis',(-1.4081690688991E-16,-6.98296267768627E-15,
1.));
#129865=DIRECTION('ref_axis',(-1.,7.99858039355471E-31,-1.4081690688991E-16));
#129866=DIRECTION('center_axis',(-1.4081690688991E-16,-6.98296267768627E-15,
1.));
#129867=DIRECTION('ref_axis',(-1.,7.99858039355471E-31,-1.4081690688991E-16));
#129868=DIRECTION('',(-0.404509815527948,-0.293899304131707,-0.86602252174666));
#129869=DIRECTION('center_axis',(-1.4081690688991E-16,-6.98296267768627E-15,
1.));
#129870=DIRECTION('ref_axis',(-1.,9.83319205199467E-31,-1.40816906889911E-16));
#129871=DIRECTION('',(0.743144825477393,0.669130606358859,4.77716140639646E-15));
#129872=DIRECTION('center_axis',(1.4081690688991E-16,6.98296267768627E-15,
-1.));
#129873=DIRECTION('ref_axis',(-1.,1.06581410364015E-14,-1.40816906889836E-16));
#129874=DIRECTION('',(-0.809016994374947,-0.587785252292474,-4.21840575002201E-15));
#129875=DIRECTION('center_axis',(-1.4081690688991E-16,-6.98296267768627E-15,
1.));
#129876=DIRECTION('ref_axis',(-1.,8.32577322149061E-31,-1.39145123902276E-16));
#129877=DIRECTION('center_axis',(-0.668334867928916,0.743860540860037,-7.86457174434936E-6));
#129878=DIRECTION('ref_axis',(-4.16662513155882E-6,6.82906352319985E-6,
0.999999999968002));
#129879=DIRECTION('center_axis',(0.588650770899605,-0.808387450333965,-7.86457259917611E-6));
#129880=DIRECTION('ref_axis',(-0.68554633998471,-0.499205608625405,0.529924500330479));
#129881=DIRECTION('center_axis',(-1.4081690688991E-16,-6.98296267768627E-15,
1.));
#129882=DIRECTION('ref_axis',(-1.,8.07722881720021E-31,-1.42096112075504E-16));
#129883=DIRECTION('center_axis',(-0.668368793156571,0.743830058708953,9.77059567102182E-6));
#129884=DIRECTION('ref_axis',(0.650581635231353,0.584586753101783,-0.484769908304563));
#129885=DIRECTION('center_axis',(0.58861390137142,-0.808414296643035,9.77052095728339E-6));
#129886=DIRECTION('ref_axis',(0.707081738813595,0.51482687314892,-0.484756336028781));
#129887=DIRECTION('center_axis',(-1.4081690688991E-16,-6.98296267768627E-15,
1.));
#129888=DIRECTION('ref_axis',(-1.,8.24049048117772E-31,-1.37719829560012E-16));
#129889=DIRECTION('center_axis',(0.671059269896725,-0.74140370646214,-1.81624800062407E-5));
#129890=DIRECTION('ref_axis',(0.64150184440888,0.58062382187108,0.501349539838051));
#129891=DIRECTION('center_axis',(-0.585681203637433,0.810541502562979,-1.81316453546949E-5));
#129892=DIRECTION('ref_axis',(0.702719177033075,0.507782078836375,0.498340364251751));
#129893=DIRECTION('center_axis',(-1.4081690688991E-16,-6.98296267768627E-15,
1.));
#129894=DIRECTION('ref_axis',(-1.,8.26087817385229E-31,-1.38060560438432E-16));
#129895=DIRECTION('center_axis',(0.671069287653591,-0.741394639059436,-1.84940662719067E-5));
#129896=DIRECTION('ref_axis',(0.642769650610767,0.581811851822409,-0.498339387699479));
#129897=DIRECTION('center_axis',(-0.585670251949389,0.810549415913883,-1.85257117335253E-5));
#129898=DIRECTION('ref_axis',(0.701329627215442,0.506740987740792,-0.501348506862578));
#129899=DIRECTION('center_axis',(-1.4081690688991E-16,-6.98296267768627E-15,
1.));
#129900=DIRECTION('ref_axis',(-1.,9.83319205199467E-31,-1.40816906889911E-16));
#129901=DIRECTION('center_axis',(-1.4081690688991E-16,-6.98296267768627E-15,
1.));
#129902=DIRECTION('ref_axis',(-1.,8.46073526001725E-31,-1.4081690688991E-16));
#129903=DIRECTION('',(0.809016994374947,0.587785252292474,4.21840575002201E-15));
#129904=DIRECTION('center_axis',(-1.4081690688991E-16,-6.98296267768627E-15,
1.));
#129905=DIRECTION('ref_axis',(-1.,7.97077743482043E-31,-1.4081690688991E-16));
#129906=DIRECTION('center_axis',(-1.4081690688991E-16,-6.98296267768627E-15,
1.));
#129907=DIRECTION('ref_axis',(-1.,7.97077743482043E-31,-1.4081690688991E-16));
#129908=DIRECTION('center_axis',(-1.4081690688991E-16,-6.98296267768627E-15,
1.));
#129909=DIRECTION('ref_axis',(-1.,7.97077743482043E-31,-1.4081690688991E-16));
#129910=DIRECTION('',(-0.866025403784438,-0.500000000000001,-3.61343235749215E-15));
#129911=DIRECTION('center_axis',(1.4081690688991E-16,6.98296267768627E-15,
-1.));
#129912=DIRECTION('ref_axis',(1.,-7.97077743482043E-31,1.4081690688991E-16));
#129913=DIRECTION('',(0.404509888559913,0.293899542971726,-0.866022406579794));
#129914=DIRECTION('center_axis',(1.4081690688991E-16,6.98296267768627E-15,
-1.));
#129915=DIRECTION('ref_axis',(-1.,7.97577417048809E-31,-1.40816906889911E-16));
#129916=DIRECTION('',(-0.433019586648905,-0.249998457755607,0.866022406579778));
#129917=DIRECTION('center_axis',(-1.4081690688991E-16,-6.98296267768627E-15,
1.));
#129918=DIRECTION('ref_axis',(-1.,9.83319205199467E-31,-1.40816906889911E-16));
#129919=DIRECTION('center_axis',(-1.4081690688991E-16,-6.98296267768627E-15,
1.));
#129920=DIRECTION('ref_axis',(-1.,7.98248735348668E-31,-1.4081690688991E-16));
#129921=DIRECTION('',(0.809016994374947,0.587785252292474,4.21840575002201E-15));
#129922=DIRECTION('center_axis',(1.4081690688991E-16,6.98296267768627E-15,
-1.));
#129923=DIRECTION('ref_axis',(-1.,7.98707387273907E-31,-1.4081690688991E-16));
#129924=DIRECTION('',(-0.866025403784438,-0.500000000000001,-3.61343235749215E-15));
#129925=DIRECTION('center_axis',(-1.4081690688991E-16,-6.98296267768627E-15,
1.));
#129926=DIRECTION('ref_axis',(-1.,7.99150043815584E-31,-1.4081690688991E-16));
#129927=DIRECTION('center_axis',(-1.4081690688991E-16,-6.98296267768627E-15,
1.));
#129928=DIRECTION('ref_axis',(1.,-7.99370576998456E-31,1.4081690688991E-16));
#129929=DIRECTION('',(0.40451525571868,0.293891816351526,0.866022521746664));
#129930=DIRECTION('center_axis',(-1.4081690688991E-16,-6.98296267768627E-15,
1.));
#129931=DIRECTION('ref_axis',(-1.,7.99858039355471E-31,-1.4081690688991E-16));
#129932=DIRECTION('center_axis',(-1.4081690688991E-16,-6.98296267768627E-15,
1.));
#129933=DIRECTION('ref_axis',(-1.,7.99858039355471E-31,-1.4081690688991E-16));
#129934=DIRECTION('center_axis',(-1.4081690688991E-16,-6.98296267768627E-15,
1.));
#129935=DIRECTION('ref_axis',(-1.,7.99858039355471E-31,-1.4081690688991E-16));
#129936=DIRECTION('',(-0.433014711050233,-0.250006503598672,-0.866022521746663));
#129937=DIRECTION('center_axis',(-1.4081690688991E-16,-6.98296267768627E-15,
1.));
#129938=DIRECTION('ref_axis',(-1.,9.83319205199467E-31,-1.40816906889911E-16));
#129939=DIRECTION('',(0.809016994374947,0.587785252292474,4.21840575002201E-15));
#129940=DIRECTION('center_axis',(1.4081690688991E-16,6.98296267768627E-15,
-1.));
#129941=DIRECTION('ref_axis',(-1.,1.24344978758018E-14,-1.40816906889824E-16));
#129942=DIRECTION('',(-0.866025403784438,-0.500000000000001,-3.61343235749215E-15));
#129943=DIRECTION('center_axis',(-1.4081690688991E-16,-6.98296267768627E-15,
1.));
#129944=DIRECTION('ref_axis',(-1.,8.32577322149061E-31,-1.39145123902276E-16));
#129945=DIRECTION('center_axis',(-0.586919060371807,0.809645611678606,-7.86457181291262E-6));
#129946=DIRECTION('ref_axis',(-3.4299684487921E-6,7.2271841840149E-6,0.999999999968002));
#129947=DIRECTION('center_axis',(0.500926582476734,-0.865489779781557,-7.86457237844701E-6));
#129948=DIRECTION('ref_axis',(-0.733972040528689,-0.424811802651091,0.529924500330455));
#129949=DIRECTION('center_axis',(-1.4081690688991E-16,-6.98296267768627E-15,
1.));
#129950=DIRECTION('ref_axis',(-1.,8.07722881720021E-31,-1.42096112075504E-16));
#129951=DIRECTION('center_axis',(-0.586955986007611,0.809618842662625,9.77059194293215E-6));
#129952=DIRECTION('ref_axis',(0.708123635910574,0.513380027141175,-0.484769908304254));
#129953=DIRECTION('center_axis',(0.500887108717654,-0.865512625110117,9.77051538527543E-6));
#129954=DIRECTION('ref_axis',(0.757022332966266,0.438096430108902,-0.484756336024758));
#129955=DIRECTION('center_axis',(-1.4081690688991E-16,-6.98296267768627E-15,
1.));
#129956=DIRECTION('ref_axis',(-1.,8.24049048117772E-31,-1.37719829560012E-16));
#129957=DIRECTION('center_axis',(0.589885346904554,-0.807487013627723,-1.81624797025065E-5));
#129958=DIRECTION('ref_axis',(0.698679346016,0.510387901840437,0.50134953984777));
#129959=DIRECTION('center_axis',(-0.497748123045552,0.867321627584527,-1.81316453185413E-5));
#129960=DIRECTION('ref_axis',(0.75194728823168,0.431546239795302,0.498340364248732));
#129961=DIRECTION('center_axis',(-1.4081690688991E-16,-6.98296267768627E-15,
1.));
#129962=DIRECTION('ref_axis',(-1.,8.26087817385229E-31,-1.38060560438432E-16));
#129963=DIRECTION('center_axis',(0.589896257574276,-0.807479043045597,-1.84940891229696E-5));
#129964=DIRECTION('ref_axis',(0.700064389991712,0.511436901808062,-0.498339387701296));
#129965=DIRECTION('center_axis',(-0.497736404184271,0.867328352820608,-1.85257173268874E-5));
#129966=DIRECTION('ref_axis',(0.75045652685783,0.430656099410795,-0.501348506865995));
#129967=DIRECTION('center_axis',(-1.4081690688991E-16,-6.98296267768627E-15,
1.));
#129968=DIRECTION('ref_axis',(-1.,9.83319205199467E-31,-1.40816906889911E-16));
#129969=DIRECTION('center_axis',(-1.4081690688991E-16,-6.98296267768627E-15,
1.));
#129970=DIRECTION('ref_axis',(-1.,8.46073526001725E-31,-1.4081690688991E-16));
#129971=DIRECTION('',(0.866025403784438,0.500000000000001,3.61343235749215E-15));
#129972=DIRECTION('center_axis',(-1.4081690688991E-16,-6.98296267768627E-15,
1.));
#129973=DIRECTION('ref_axis',(-1.,7.97077743482043E-31,-1.4081690688991E-16));
#129974=DIRECTION('center_axis',(-1.4081690688991E-16,-6.98296267768627E-15,
1.));
#129975=DIRECTION('ref_axis',(-1.,7.97077743482043E-31,-1.4081690688991E-16));
#129976=DIRECTION('center_axis',(-1.4081690688991E-16,-6.98296267768627E-15,
1.));
#129977=DIRECTION('ref_axis',(-1.,7.97077743482043E-31,-1.4081690688991E-16));
#129978=DIRECTION('',(-0.913545457642601,-0.406736643075801,-2.96886944389428E-15));
#129979=DIRECTION('center_axis',(1.4081690688991E-16,6.98296267768627E-15,
-1.));
#129980=DIRECTION('ref_axis',(1.,-7.97077743482043E-31,1.4081690688991E-16));
#129981=DIRECTION('',(0.43301480864772,0.250006733496374,-0.86602240657979));
#129982=DIRECTION('center_axis',(1.4081690688991E-16,6.98296267768627E-15,
-1.));
#129983=DIRECTION('ref_axis',(-1.,7.97577417048809E-31,-1.40816906889911E-16));
#129984=DIRECTION('',(-0.456779414654134,-0.203366068089034,0.866022406579779));
#129985=DIRECTION('center_axis',(-1.4081690688991E-16,-6.98296267768627E-15,
1.));
#129986=DIRECTION('ref_axis',(-1.,9.83319205199467E-31,-1.40816906889911E-16));
#129987=DIRECTION('center_axis',(-1.4081690688991E-16,-6.98296267768627E-15,
1.));
#129988=DIRECTION('ref_axis',(-1.,7.98248735348668E-31,-1.4081690688991E-16));
#129989=DIRECTION('',(0.866025403784438,0.500000000000001,3.61343235749215E-15));
#129990=DIRECTION('center_axis',(1.4081690688991E-16,6.98296267768627E-15,
-1.));
#129991=DIRECTION('ref_axis',(-1.,-1.24344978758018E-14,-1.40816906889997E-16));
#129992=DIRECTION('',(-0.913545457642601,-0.406736643075801,-2.96886944389428E-15));
#129993=DIRECTION('center_axis',(-1.4081690688991E-16,-6.98296267768627E-15,
1.));
#129994=DIRECTION('ref_axis',(-1.,7.99150043815584E-31,-1.4081690688991E-16));
#129995=DIRECTION('center_axis',(-1.4081690688991E-16,-6.98296267768627E-15,
1.));
#129996=DIRECTION('ref_axis',(1.,-7.99370576998456E-31,1.4081690688991E-16));
#129997=DIRECTION('',(0.433019338752905,0.249998488182556,0.866022521746654));
#129998=DIRECTION('center_axis',(-1.4081690688991E-16,-6.98296267768627E-15,
1.));
#129999=DIRECTION('ref_axis',(-1.,7.99858039355471E-31,-1.4081690688991E-16));
#130000=DIRECTION('center_axis',(-1.4081690688991E-16,-6.98296267768627E-15,
1.));
#130001=DIRECTION('ref_axis',(-1.,7.99858039355471E-31,-1.4081690688991E-16));
#130002=DIRECTION('center_axis',(-1.4081690688991E-16,-6.98296267768627E-15,
1.));
#130003=DIRECTION('ref_axis',(-1.,7.99858039355471E-31,-1.4081690688991E-16));
#130004=DIRECTION('',(-0.456775406784136,-0.203374579494979,-0.86602252174665));
#130005=DIRECTION('center_axis',(-1.4081690688991E-16,-6.98296267768627E-15,
1.));
#130006=DIRECTION('ref_axis',(-1.,9.83319205199467E-31,-1.40816906889911E-16));
#130007=DIRECTION('',(0.866025403784438,0.500000000000001,3.61343235749215E-15));
#130008=DIRECTION('center_axis',(1.4081690688991E-16,6.98296267768627E-15,
-1.));
#130009=DIRECTION('ref_axis',(-1.,8.01265634860448E-31,-1.4081690688991E-16));
#130010=DIRECTION('',(-0.913545457642601,-0.406736643075801,-2.96886944389428E-15));
#130011=DIRECTION('center_axis',(-1.4081690688991E-16,-6.98296267768627E-15,
1.));
#130012=DIRECTION('ref_axis',(-1.,8.32577322149061E-31,-1.39145123902276E-16));
#130013=DIRECTION('center_axis',(-0.499072844768457,0.866560035746438,-7.86457193853739E-6));
#130014=DIRECTION('ref_axis',(-2.65573230665241E-6,7.54612235481617E-6,
0.999999999968002));
#130015=DIRECTION('center_axis',(0.4077141375907,-0.913109622086428,-7.86457248217639E-6));
#130016=DIRECTION('ref_axis',(-0.774356189802968,-0.34576366966955,0.529924500330449));
#130017=DIRECTION('center_axis',(-1.4081690688991E-16,-6.98296267768627E-15,
1.));
#130018=DIRECTION('ref_axis',(-1.,8.07722881720021E-31,-1.42096112075504E-16));
#130019=DIRECTION('center_axis',(-0.499112366248239,0.866537273152528,9.77058724011587E-6));
#130020=DIRECTION('ref_axis',(0.757907285850955,0.436548602171837,-0.484769908302748));
#130021=DIRECTION('center_axis',(0.407672492086805,-0.913128216134115,9.77051721567626E-6));
#130022=DIRECTION('ref_axis',(0.798668832019429,0.356566110901419,-0.484756336026007));
#130023=DIRECTION('center_axis',(-1.4081690688991E-16,-6.98296267768627E-15,
1.));
#130024=DIRECTION('ref_axis',(-1.,8.24049048117772E-31,-1.37719829560012E-16));
#130025=DIRECTION('center_axis',(0.502248516610505,-0.864723324094286,-1.81624798863006E-5));
#130026=DIRECTION('ref_axis',(0.74820197050765,0.434560065157462,0.50134953984103));
#130027=DIRECTION('center_axis',(-0.40436160985703,0.91459919535558,-1.81316453178961E-5));
#130028=DIRECTION('ref_axis',(0.792936907585205,0.350582289843673,0.498340364246343));
#130029=DIRECTION('center_axis',(-1.4081690688991E-16,-6.98296267768627E-15,
1.));
#130030=DIRECTION('ref_axis',(-1.,8.26087817385229E-31,-1.38060560438432E-16));
#130031=DIRECTION('center_axis',(0.502260200678538,-0.864716537642437,-1.84940579829993E-5));
#130032=DIRECTION('ref_axis',(0.74968907742253,0.435458542075418,-0.498339387693675));
#130033=DIRECTION('center_axis',(-0.404349252215686,0.914604658794943,-1.85257198772365E-5));
#130034=DIRECTION('ref_axis',(0.791361267751807,0.349852852736935,-0.501348506863321));
#130035=DIRECTION('center_axis',(-1.4081690688991E-16,-6.98296267768627E-15,
1.));
#130036=DIRECTION('ref_axis',(-1.,9.83319205199467E-31,-1.40816906889911E-16));
#130037=DIRECTION('center_axis',(-1.4081690688991E-16,-6.98296267768627E-15,
1.));
#130038=DIRECTION('ref_axis',(-1.,8.46073526001725E-31,-1.4081690688991E-16));
#130039=DIRECTION('',(0.913545457642601,0.406736643075801,2.96886944389428E-15));
#130040=DIRECTION('center_axis',(-1.4081690688991E-16,-6.98296267768627E-15,
1.));
#130041=DIRECTION('ref_axis',(-1.,7.97077743482043E-31,-1.4081690688991E-16));
#130042=DIRECTION('center_axis',(-1.4081690688991E-16,-6.98296267768627E-15,
1.));
#130043=DIRECTION('ref_axis',(-1.,7.97077743482043E-31,-1.4081690688991E-16));
#130044=DIRECTION('center_axis',(-1.4081690688991E-16,-6.98296267768627E-15,
1.));
#130045=DIRECTION('ref_axis',(-1.,7.97077743482043E-31,-1.4081690688991E-16));
#130046=DIRECTION('',(-0.951056516295153,-0.309016994374948,-2.29177897539323E-15));
#130047=DIRECTION('center_axis',(1.4081690688991E-16,6.98296267768627E-15,
-1.));
#130048=DIRECTION('ref_axis',(1.,-7.97077743482043E-31,1.4081690688991E-16));
#130049=DIRECTION('',(0.456775527877823,0.203374797931579,-0.866022406579775));
#130050=DIRECTION('center_axis',(1.4081690688991E-16,6.98296267768627E-15,
-1.));
#130051=DIRECTION('ref_axis',(-1.,7.97577417048809E-31,-1.40816906889911E-16));
#130052=DIRECTION('',(-0.475534671805145,-0.154505557223411,0.866022406579793));
#130053=DIRECTION('center_axis',(-1.4081690688991E-16,-6.98296267768627E-15,
1.));
#130054=DIRECTION('ref_axis',(-1.,9.83319205199467E-31,-1.40816906889911E-16));
#130055=DIRECTION('center_axis',(-1.4081690688991E-16,-6.98296267768627E-15,
1.));
#130056=DIRECTION('ref_axis',(-1.,7.98248735348668E-31,-1.4081690688991E-16));
#130057=DIRECTION('',(0.9135454576426,0.406736643075801,2.96886944389428E-15));
#130058=DIRECTION('center_axis',(1.4081690688991E-16,6.98296267768627E-15,
-1.));
#130059=DIRECTION('ref_axis',(-1.,1.24344978758018E-14,-1.40816906889824E-16));
#130060=DIRECTION('',(-0.951056516295153,-0.309016994374948,-2.29177897539323E-15));
#130061=DIRECTION('center_axis',(-1.4081690688991E-16,-6.98296267768627E-15,
1.));
#130062=DIRECTION('ref_axis',(-1.,7.99150043815584E-31,-1.4081690688991E-16));
#130063=DIRECTION('center_axis',(-1.4081690688991E-16,-6.98296267768627E-15,
1.));
#130064=DIRECTION('ref_axis',(1.,-7.99370576998456E-31,1.4081690688991E-16));
#130065=DIRECTION('',(0.456779171296638,0.203366124261504,0.866022521746641));
#130066=DIRECTION('center_axis',(-1.4081690688991E-16,-6.98296267768627E-15,
1.));
#130067=DIRECTION('ref_axis',(-1.,7.99858039355471E-31,-1.4081690688991E-16));
#130068=DIRECTION('center_axis',(-1.4081690688991E-16,-6.98296267768627E-15,
1.));
#130069=DIRECTION('ref_axis',(-1.,7.99858039355471E-31,-1.4081690688991E-16));
#130070=DIRECTION('center_axis',(-1.4081690688991E-16,-6.98296267768627E-15,
1.));
#130071=DIRECTION('ref_axis',(-1.,7.99858039355471E-31,-1.4081690688991E-16));
#130072=DIRECTION('',(-0.47553157557488,-0.154514440939479,-0.866022521746653));
#130073=DIRECTION('center_axis',(-1.4081690688991E-16,-6.98296267768627E-15,
1.));
#130074=DIRECTION('ref_axis',(-1.,9.83319205199467E-31,-1.40816906889911E-16));
#130075=DIRECTION('',(0.913545457642601,0.406736643075801,2.96886944389428E-15));
#130076=DIRECTION('center_axis',(1.4081690688991E-16,6.98296267768627E-15,
-1.));
#130077=DIRECTION('ref_axis',(-1.,1.24344978758018E-14,-1.40816906889824E-16));
#130078=DIRECTION('',(-0.951056516295153,-0.309016994374948,-2.29177897539323E-15));
#130079=DIRECTION('center_axis',(-1.4081690688991E-16,-6.98296267768627E-15,
1.));
#130080=DIRECTION('ref_axis',(-1.,8.32577322149061E-31,-1.39145123902276E-16));
#130081=DIRECTION('center_axis',(-0.405758682640331,0.913980246723162,-7.86457182175925E-6));
#130082=DIRECTION('ref_axis',(-1.85239931600469E-6,7.78238341415138E-6,
0.999999999968001));
#130083=DIRECTION('center_axis',(0.310034691293513,-0.950725244291265,-7.86457232249133E-6));
#130084=DIRECTION('ref_axis',(-0.806256330617362,-0.262927277567242,0.529924500330477));
#130085=DIRECTION('center_axis',(-1.4081690688991E-16,-6.98296267768627E-15,
1.));
#130086=DIRECTION('ref_axis',(-1.,8.07722881720021E-31,-1.42096112075504E-16));
#130087=DIRECTION('center_axis',(-0.405800366958868,0.913961739943519,9.77058183081883E-6));
#130088=DIRECTION('ref_axis',(0.799387144964317,0.35493425936279,-0.484769908303295));
#130089=DIRECTION('center_axis',(0.309991330319623,-0.950739383338677,9.77051486152074E-6));
#130090=DIRECTION('ref_axis',(0.831564948217564,0.271129178767091,-0.484756336025639));
#130091=DIRECTION('center_axis',(-1.4081690688991E-16,-6.98296267768627E-15,
1.));
#130092=DIRECTION('ref_axis',(-1.,8.24049048117772E-31,-1.37719829560012E-16));
#130093=DIRECTION('center_axis',(0.409108946466101,-0.912485544867162,-1.81624798278693E-5));
#130094=DIRECTION('ref_axis',(0.78952713763448,0.353971097460131,0.501349539843786));
#130095=DIRECTION('center_axis',(-0.306544826252812,0.951856222950124,-1.81316452657696E-5));
#130096=DIRECTION('ref_axis',(0.825238944242273,0.265777286958772,0.498340364251916));
#130097=DIRECTION('center_axis',(-1.4081690688991E-16,-6.98296267768627E-15,
1.));
#130098=DIRECTION('ref_axis',(-1.,8.26087817385229E-31,-1.38060560438432E-16));
#130099=DIRECTION('center_axis',(0.409121275899175,-0.91248001691248,-1.84940690708923E-5));
#130100=DIRECTION('ref_axis',(0.791100014432547,0.354709207426512,-0.498339387698464));
#130101=DIRECTION('center_axis',(-0.306531965213273,0.951860364738068,-1.85257020962267E-5));
#130102=DIRECTION('ref_axis',(0.823595688993123,0.265216544996729,-0.501348506861187));
#130103=DIRECTION('center_axis',(-1.4081690688991E-16,-6.98296267768627E-15,
1.));
#130104=DIRECTION('ref_axis',(-1.,9.83319205199467E-31,-1.40816906889911E-16));
#130105=DIRECTION('center_axis',(-1.4081690688991E-16,-6.98296267768627E-15,
1.));
#130106=DIRECTION('ref_axis',(-1.,8.46073526001725E-31,-1.4081690688991E-16));
#130107=DIRECTION('',(0.951056516295153,0.309016994374948,2.29177897539323E-15));
#130108=DIRECTION('center_axis',(-1.4081690688991E-16,-6.98296267768627E-15,
1.));
#130109=DIRECTION('ref_axis',(-1.,7.97077743482043E-31,-1.4081690688991E-16));
#130110=DIRECTION('center_axis',(-1.4081690688991E-16,-6.98296267768627E-15,
1.));
#130111=DIRECTION('ref_axis',(-1.,7.97077743482043E-31,-1.4081690688991E-16));
#130112=DIRECTION('center_axis',(-1.4081690688991E-16,-6.98296267768627E-15,
1.));
#130113=DIRECTION('ref_axis',(-1.,7.97077743482043E-31,-1.4081690688991E-16));
#130114=DIRECTION('',(-0.978147600733806,-0.20791169081776,-1.58957929685218E-15));
#130115=DIRECTION('center_axis',(1.4081690688991E-16,6.98296267768627E-15,
-1.));
#130116=DIRECTION('ref_axis',(1.,-7.97077743482043E-31,1.4081690688991E-16));
#130117=DIRECTION('',(0.475531718838049,0.154514645521708,-0.866022406579779));
#130118=DIRECTION('center_axis',(1.4081690688991E-16,6.98296267768627E-15,
-1.));
#130119=DIRECTION('ref_axis',(-1.,7.97577417048809E-31,-1.40816906889911E-16));
#130120=DIRECTION('',(-0.489079871579875,-0.103952251140501,0.866022406579781));
#130121=DIRECTION('center_axis',(-1.4081690688991E-16,-6.98296267768627E-15,
1.));
#130122=DIRECTION('ref_axis',(-1.,9.83319205199467E-31,-1.40816906889911E-16));
#130123=DIRECTION('center_axis',(-1.4081690688991E-16,-6.98296267768627E-15,
1.));
#130124=DIRECTION('ref_axis',(-1.,7.98248735348668E-31,-1.4081690688991E-16));
#130125=DIRECTION('',(0.951056516295153,0.309016994374948,2.29177897539323E-15));
#130126=DIRECTION('center_axis',(1.4081690688991E-16,6.98296267768627E-15,
-1.));
#130127=DIRECTION('ref_axis',(-1.,7.98707387273907E-31,-1.4081690688991E-16));
#130128=DIRECTION('',(-0.978147600733806,-0.20791169081776,-1.58957929685218E-15));
#130129=DIRECTION('center_axis',(-1.4081690688991E-16,-6.98296267768627E-15,
1.));
#130130=DIRECTION('ref_axis',(-1.,7.99150043815584E-31,-1.4081690688991E-16));
#130131=DIRECTION('center_axis',(-1.4081690688991E-16,-6.98296267768627E-15,
1.));
#130132=DIRECTION('ref_axis',(1.,-7.99370576998456E-31,1.4081690688991E-16));
#130133=DIRECTION('',(0.475534435652401,0.154505638525951,0.866022521746658));
#130134=DIRECTION('center_axis',(-1.4081690688991E-16,-6.98296267768627E-15,
1.));
#130135=DIRECTION('ref_axis',(-1.,7.99858039355471E-31,-1.4081690688991E-16));
#130136=DIRECTION('center_axis',(-1.4081690688991E-16,-6.98296267768627E-15,
1.));
#130137=DIRECTION('ref_axis',(-1.,7.99858039355471E-31,-1.4081690688991E-16));
#130138=DIRECTION('center_axis',(-1.4081690688991E-16,-6.98296267768627E-15,
1.));
#130139=DIRECTION('ref_axis',(-1.,7.99858039355471E-31,-1.4081690688991E-16));
#130140=DIRECTION('',(-0.489077720912241,-0.103961409834797,-0.866022521746663));
#130141=DIRECTION('center_axis',(-1.4081690688991E-16,-6.98296267768627E-15,
1.));
#130142=DIRECTION('ref_axis',(-1.,9.83319205199467E-31,-1.40816906889911E-16));
#130143=DIRECTION('',(0.951056516295153,0.309016994374948,2.29177897539323E-15));
#130144=DIRECTION('center_axis',(1.4081690688991E-16,6.98296267768627E-15,
-1.));
#130145=DIRECTION('ref_axis',(-1.,1.33226762955019E-14,-1.40816906889817E-16));
#130146=DIRECTION('',(-0.978147600733806,-0.20791169081776,-1.58957929685218E-15));
#130147=DIRECTION('center_axis',(-1.4081690688991E-16,-6.98296267768627E-15,
1.));
#130148=DIRECTION('ref_axis',(-1.,8.32577322149061E-31,-1.39145123902276E-16));
#130149=DIRECTION('center_axis',(-0.307998943474451,0.951386698854241,-7.86457217331017E-6));
#130150=DIRECTION('ref_axis',(-1.02877118498542E-6,7.93337950118864E-6,
0.999999999968002));
#130151=DIRECTION('center_axis',(0.208958440039605,-0.977924521767587,-7.86457232448164E-6));
#130152=DIRECTION('ref_axis',(-0.829322958353508,-0.177210199190942,0.529924500330464));
#130153=DIRECTION('center_axis',(-1.4081690688991E-16,-6.98296267768627E-15,
1.));
#130154=DIRECTION('ref_axis',(-1.,8.07722881720021E-31,-1.42096112075504E-16));
#130155=DIRECTION('center_axis',(-0.308042333920874,0.951372650656469,9.77059417868512E-6));
#130156=DIRECTION('ref_axis',(0.83210875123558,0.269431182533746,-0.484769908302517));
#130157=DIRECTION('center_axis',(0.208913838670284,-0.977934050903528,9.77051762784349E-6));
#130158=DIRECTION('ref_axis',(0.855350264826107,0.182721698612545,-0.484756336026725));
#130159=DIRECTION('center_axis',(-1.4081690688991E-16,-6.98296267768627E-15,
1.));
#130160=DIRECTION('ref_axis',(-1.,8.24049048117772E-31,-1.37719829560012E-16));
#130161=DIRECTION('center_axis',(0.311487093092632,-0.950250383060605,-1.81624797870643E-5));
#130162=DIRECTION('ref_axis',(0.822202080224617,0.26950394834691,0.501349539841953));
#130163=DIRECTION('center_axis',(-0.205369473383596,0.978684514577291,-1.81316452352081E-5));
#130164=DIRECTION('ref_axis',(0.848499490339199,0.178060372502337,0.498340364247618));
#130165=DIRECTION('center_axis',(-1.4081690688991E-16,-6.98296267768627E-15,
1.));
#130166=DIRECTION('ref_axis',(-1.,8.26087817385229E-31,-1.38060560438432E-16));
#130167=DIRECTION('center_axis',(0.311499932819129,-0.950246174163121,-1.84940568302248E-5));
#130168=DIRECTION('ref_axis',(0.823843494140198,0.270073604475308,-0.498339387695358));
#130169=DIRECTION('center_axis',(-0.205356249869677,0.978687289330081,-1.85257132684071E-5));
#130170=DIRECTION('ref_axis',(0.84680662351654,0.177674469288859,-0.501348506860686));
#130171=DIRECTION('center_axis',(-1.4081690688991E-16,-6.98296267768627E-15,
1.));
#130172=DIRECTION('ref_axis',(-1.,9.83319205199467E-31,-1.40816906889911E-16));
#130173=DIRECTION('center_axis',(-1.4081690688991E-16,-6.98296267768627E-15,
1.));
#130174=DIRECTION('ref_axis',(-1.,8.46073526001725E-31,-1.4081690688991E-16));
#130175=DIRECTION('',(0.978147600733806,0.20791169081776,1.58957929685218E-15));
#130176=DIRECTION('center_axis',(-1.4081690688991E-16,-6.98296267768627E-15,
1.));
#130177=DIRECTION('ref_axis',(-1.,7.97077743482043E-31,-1.4081690688991E-16));
#130178=DIRECTION('center_axis',(-1.4081690688991E-16,-6.98296267768627E-15,
1.));
#130179=DIRECTION('ref_axis',(-1.,7.97077743482043E-31,-1.4081690688991E-16));
#130180=DIRECTION('center_axis',(-1.4081690688991E-16,-6.98296267768627E-15,
1.));
#130181=DIRECTION('ref_axis',(-1.,7.97077743482043E-31,-1.4081690688991E-16));
#130182=DIRECTION('',(-0.994521895368273,-0.104528463267654,-8.69963854893977E-16));
#130183=DIRECTION('center_axis',(1.4081690688991E-16,6.98296267768627E-15,
-1.));
#130184=DIRECTION('ref_axis',(1.,-7.97077743482043E-31,1.4081690688991E-16));
#130185=DIRECTION('',(0.48907788477527,0.103961598321241,-0.866022406579784));
#130186=DIRECTION('center_axis',(1.4081690688991E-16,6.98296267768627E-15,
-1.));
#130187=DIRECTION('ref_axis',(-1.,7.97577417048809E-31,-1.40816906889911E-16));
#130188=DIRECTION('',(-0.497266609935059,-0.0522600224406523,0.866022406579758));
#130189=DIRECTION('center_axis',(-1.4081690688991E-16,-6.98296267768627E-15,
1.));
#130190=DIRECTION('ref_axis',(-1.,9.83319205199467E-31,-1.40816906889911E-16));
#130191=DIRECTION('center_axis',(-1.4081690688991E-16,-6.98296267768627E-15,
1.));
#130192=DIRECTION('ref_axis',(-1.,7.98248735348668E-31,-1.4081690688991E-16));
#130193=DIRECTION('',(0.978147600733806,0.20791169081776,1.58957929685218E-15));
#130194=DIRECTION('center_axis',(1.4081690688991E-16,6.98296267768627E-15,
-1.));
#130195=DIRECTION('ref_axis',(-1.,7.98707387273907E-31,-1.4081690688991E-16));
#130196=DIRECTION('',(-0.994521895368273,-0.104528463267654,-8.69963854893977E-16));
#130197=DIRECTION('center_axis',(-1.4081690688991E-16,-6.98296267768627E-15,
1.));
#130198=DIRECTION('ref_axis',(-1.,7.99150043815584E-31,-1.4081690688991E-16));
#130199=DIRECTION('center_axis',(-1.4081690688991E-16,-6.98296267768627E-15,
1.));
#130200=DIRECTION('ref_axis',(1.,-7.99370576998456E-31,1.4081690688991E-16));
#130201=DIRECTION('',(0.489079645219225,0.103952356682307,0.866022521746653));
#130202=DIRECTION('center_axis',(-1.4081690688991E-16,-6.98296267768627E-15,
1.));
#130203=DIRECTION('ref_axis',(-1.,7.99858039355471E-31,-1.4081690688991E-16));
#130204=DIRECTION('center_axis',(-1.4081690688991E-16,-6.98296267768627E-15,
1.));
#130205=DIRECTION('ref_axis',(-1.,7.99858039355471E-31,-1.4081690688991E-16));
#130206=DIRECTION('center_axis',(-1.4081690688991E-16,-6.98296267768627E-15,
1.));
#130207=DIRECTION('ref_axis',(-1.,7.99858039355471E-31,-1.4081690688991E-16));
#130208=DIRECTION('',(-0.497265428393217,-0.052269355768654,-0.866022521746658));
#130209=DIRECTION('center_axis',(-1.4081690688991E-16,-6.98296267768627E-15,
1.));
#130210=DIRECTION('ref_axis',(-1.,9.83319205199467E-31,-1.40816906889911E-16));
#130211=DIRECTION('',(0.978147600733806,0.20791169081776,1.58957929685218E-15));
#130212=DIRECTION('center_axis',(1.4081690688991E-16,6.98296267768627E-15,
-1.));
#130213=DIRECTION('ref_axis',(-1.,8.01265634860448E-31,-1.4081690688991E-16));
#130214=DIRECTION('',(-0.994521895368273,-0.104528463267654,-8.69963854893977E-16));
#130215=DIRECTION('center_axis',(-1.4081690688991E-16,-6.98296267768627E-15,
1.));
#130216=DIRECTION('ref_axis',(-1.,8.32577322149061E-31,-1.39145123902276E-16));
#130217=DIRECTION('center_axis',(-0.206864703431196,0.978369559222113,-7.86457193300846E-6));
#130218=DIRECTION('ref_axis',(-1.93871482032996E-7,7.99745524812744E-6,
0.999999999968002));
#130219=DIRECTION('center_axis',(0.10559279638925,-0.99440945353956,-7.86457230109251E-6));
#130220=DIRECTION('ref_axis',(-0.843303350210939,-0.0895515687886603,0.529924500330468));
#130221=DIRECTION('center_axis',(-1.4081690688991E-16,-6.98296267768627E-15,
1.));
#130222=DIRECTION('ref_axis',(-1.,8.07722881720021E-31,-1.42096112075504E-16));
#130223=DIRECTION('center_axis',(-0.206909324622309,0.978360123517346,9.77058376346471E-6));
#130224=DIRECTION('ref_axis',(0.85571359989698,0.180976161286345,-0.484769908304352));
#130225=DIRECTION('center_axis',(0.10554744328483,-0.994414268361317,9.77051740345421E-6));
#130226=DIRECTION('ref_axis',(0.86976418493997,0.0923122812911577,-0.484756336027217));
#130227=DIRECTION('center_axis',(-1.4081690688991E-16,-6.98296267768627E-15,
1.));
#130228=DIRECTION('ref_axis',(-1.,8.24049048117772E-31,-1.37719829560012E-16));
#130229=DIRECTION('center_axis',(0.210452521944419,-0.977604079204541,-1.81624797886102E-5));
#130230=DIRECTION('ref_axis',(0.84586880476805,0.182084057578303,0.501349539838316));
#130231=DIRECTION('center_axis',(-0.10194404958761,0.994790133859862,-1.81316452628073E-5));
#130232=DIRECTION('ref_axis',(0.862463698457381,0.0883925913424311,0.498340364248156));
#130233=DIRECTION('center_axis',(-1.4081690688991E-16,-6.98296267768627E-15,
1.));
#130234=DIRECTION('ref_axis',(-1.,8.26087817385229E-31,-1.38060560438432E-16));
#130235=DIRECTION('center_axis',(0.210465731283201,-0.977601235480703,-1.84940567325367E-5));
#130236=DIRECTION('ref_axis',(0.847560772121326,0.182479018595613,-0.498339387700273));
#130237=DIRECTION('center_axis',(-0.10193060847116,0.994791511178849,-1.85257102811266E-5));
#130238=DIRECTION('ref_axis',(0.860739767468925,0.0881857549149035,-0.501348506856886));
#130239=DIRECTION('center_axis',(-1.4081690688991E-16,-6.98296267768627E-15,
1.));
#130240=DIRECTION('ref_axis',(-1.,9.83319205199467E-31,-1.40816906889911E-16));
#130241=DIRECTION('center_axis',(-1.4081690688991E-16,-6.98296267768627E-15,
1.));
#130242=DIRECTION('ref_axis',(-1.,9.83319205199467E-31,-1.40816906889911E-16));
#130243=DIRECTION('center_axis',(-1.4081690688991E-16,-6.98296267768627E-15,
1.));
#130244=DIRECTION('ref_axis',(-1.,8.46073526001725E-31,-1.4081690688991E-16));
#130245=DIRECTION('',(0.994521895368273,0.104528463267654,8.69963854893977E-16));
#130246=DIRECTION('center_axis',(-1.4081690688991E-16,-6.98296267768627E-15,
1.));
#130247=DIRECTION('ref_axis',(-1.,7.97077743482043E-31,-1.4081690688991E-16));
#130248=DIRECTION('center_axis',(-1.4081690688991E-16,-6.98296267768627E-15,
1.));
#130249=DIRECTION('ref_axis',(-1.,7.97077743482043E-31,-1.4081690688991E-16));
#130250=DIRECTION('center_axis',(-1.4081690688991E-16,-6.98296267768627E-15,
1.));
#130251=DIRECTION('ref_axis',(-1.,7.97077743482043E-31,-1.4081690688991E-16));
#130252=DIRECTION('',(-1.,9.83319205199467E-31,-1.40816906889911E-16));
#130253=DIRECTION('center_axis',(1.4081690688991E-16,6.98296267768627E-15,
-1.));
#130254=DIRECTION('ref_axis',(1.,-7.97077743482043E-31,1.4081690688991E-16));
#130255=DIRECTION('',(0.497265611060784,0.0522695260942052,-0.866022406579779));
#130256=DIRECTION('center_axis',(1.4081690688991E-16,6.98296267768627E-15,
-1.));
#130257=DIRECTION('ref_axis',(-1.,7.97577417048809E-31,-1.40816906889911E-16));
#130258=DIRECTION('',(-0.500005191251968,4.77800115976002E-6,0.866022406579792));
#130259=DIRECTION('center_axis',(-1.4081690688991E-16,-6.98296267768627E-15,
1.));
#130260=DIRECTION('ref_axis',(-1.,9.83319205199467E-31,-1.40816906889911E-16));
#130261=DIRECTION('center_axis',(-1.4081690688991E-16,-6.98296267768627E-15,
1.));
#130262=DIRECTION('ref_axis',(-1.,7.98248735348668E-31,-1.4081690688991E-16));
#130263=DIRECTION('',(0.994521895368273,0.104528463267654,8.69963854893977E-16));
#130264=DIRECTION('center_axis',(1.4081690688991E-16,6.98296267768627E-15,
-1.));
#130265=DIRECTION('ref_axis',(-1.,7.98707387273907E-31,-1.4081690688991E-16));
#130266=DIRECTION('',(-1.,9.83319205199467E-31,-1.40816906889911E-16));
#130267=DIRECTION('center_axis',(-1.4081690688991E-16,-6.98296267768627E-15,
1.));
#130268=DIRECTION('ref_axis',(-1.,7.99150043815584E-31,-1.4081690688991E-16));
#130269=DIRECTION('center_axis',(-1.4081690688991E-16,-6.98296267768627E-15,
1.));
#130270=DIRECTION('ref_axis',(1.,-7.99370576998456E-31,1.4081690688991E-16));
#130271=DIRECTION('',(0.497266395846506,0.052260151065429,0.86602252174666));
#130272=DIRECTION('center_axis',(-1.4081690688991E-16,-6.98296267768627E-15,
1.));
#130273=DIRECTION('ref_axis',(-1.,7.99858039355471E-31,-1.4081690688991E-16));
#130274=DIRECTION('center_axis',(-1.4081690688991E-16,-6.98296267768627E-15,
1.));
#130275=DIRECTION('ref_axis',(-1.,7.99858039355471E-31,-1.4081690688991E-16));
#130276=DIRECTION('center_axis',(-1.4081690688991E-16,-6.98296267768627E-15,
1.));
#130277=DIRECTION('ref_axis',(-1.,7.99858039355471E-31,-1.4081690688991E-16));
#130278=DIRECTION('',(-0.500004991781247,-4.62770264658395E-6,-0.866022521746646));
#130279=DIRECTION('center_axis',(-1.4081690688991E-16,-6.98296267768627E-15,
1.));
#130280=DIRECTION('ref_axis',(-1.,9.83319205199467E-31,-1.40816906889911E-16));
#130281=DIRECTION('',(0.994521895368273,0.104528463267654,8.69963854893977E-16));
#130282=DIRECTION('center_axis',(1.4081690688991E-16,6.98296267768627E-15,
-1.));
#130283=DIRECTION('ref_axis',(-1.,-8.88178419700124E-16,-1.40816906889917E-16));
#130284=DIRECTION('',(-1.,9.83319205199467E-31,-1.40816906889911E-16));
#130285=DIRECTION('center_axis',(-1.4081690688991E-16,-6.98296267768627E-15,
1.));
#130286=DIRECTION('ref_axis',(-1.,9.83319205199467E-31,-1.40816906889911E-16));
#130287=DIRECTION('center_axis',(1.4081690688991E-16,6.98296267768627E-15,
-1.));
#130288=DIRECTION('ref_axis',(1.,-9.83319205199467E-31,1.40816906889911E-16));
#130289=DIRECTION('center_axis',(-1.4081690688991E-16,-6.98296267768627E-15,
1.));
#130290=DIRECTION('ref_axis',(-1.,8.32577322149061E-31,-1.39145123902276E-16));
#130291=DIRECTION('center_axis',(-0.103464010407694,0.994633197962196,-7.86457221782119E-6));
#130292=DIRECTION('ref_axis',(6.43152272453736E-7,7.97390972565421E-6,0.999999999968002));
#130293=DIRECTION('center_axis',(0.00107025596496831,-0.999999427244995,
-7.86457232244496E-6));
#130294=DIRECTION('ref_axis',(-0.848044334090886,-0.000911792658910411,
0.529924500330465));
#130295=DIRECTION('center_axis',(-1.4081690688991E-16,-6.98296267768627E-15,
1.));
#130296=DIRECTION('ref_axis',(-1.,8.07722881720021E-31,-1.42096112075504E-16));
#130297=DIRECTION('center_axis',(-0.103509373457858,0.994628478131859,9.77058599509235E-6));
#130298=DIRECTION('ref_axis',(0.869943071290751,0.0905383273446241,-0.484769908301715));
#130299=DIRECTION('center_axis',(0.00102464802302249,-0.999999475000345,
9.77051621741992E-6));
#130300=DIRECTION('ref_axis',(0.874648786634666,0.000891471298443714,-0.484756336026081));
#130301=DIRECTION('center_axis',(-1.4081690688991E-16,-6.98296267768627E-15,
1.));
#130302=DIRECTION('ref_axis',(-1.,8.24049048117772E-31,-1.37719829560012E-16));
#130303=DIRECTION('center_axis',(0.10711218892574,-0.99424694047991,-1.81624798142884E-5));
#130304=DIRECTION('ref_axis',(0.860268013667682,0.0926692157698502,0.501349539851053));
#130305=DIRECTION('center_axis',(0.00259829454877957,0.999996624262643,
-1.81316452223945E-5));
#130306=DIRECTION('ref_axis',(0.866978573811375,-0.00224363754548925,0.498340364251741));
#130307=DIRECTION('center_axis',(-1.4081690688991E-16,-6.98296267768627E-15,
1.));
#130308=DIRECTION('ref_axis',(-1.,8.26087817385229E-31,-1.38060560438432E-16));
#130309=DIRECTION('center_axis',(0.107125623152397,-0.99424549308618,-1.84940568669125E-5));
#130310=DIRECTION('ref_axis',(0.86199199692613,0.0928851544032709,-0.498339387693551));
#130311=DIRECTION('center_axis',(0.00261180600212697,0.999996589057285,
-1.85257108462124E-5));
#130312=DIRECTION('ref_axis',(0.865242466401146,-0.00226914104442312,-0.501348506864219));
#130313=DIRECTION('center_axis',(0.,-6.98296267768627E-15,1.));
#130314=DIRECTION('ref_axis',(-1.,0.,0.));
#130315=DIRECTION('',(1.,0.,0.));
#130316=DIRECTION('center_axis',(0.,6.98296267768627E-15,-1.));
#130317=DIRECTION('ref_axis',(-1.,-2.87680990140871E-12,-2.00886561723353E-26));
#130318=DIRECTION('',(-1.,0.,0.));
#130319=DIRECTION('center_axis',(0.,-6.98296267768627E-15,1.));
#130320=DIRECTION('ref_axis',(-1.,0.,0.));
#130321=DIRECTION('center_axis',(0.,-1.,-6.98296267768627E-15));
#130322=DIRECTION('ref_axis',(0.,6.98296267768627E-15,-1.));
#130323=DIRECTION('center_axis',(5.53227016421295E-17,-1.,-7.21882542163455E-15));
#130324=DIRECTION('ref_axis',(0.874651456243689,-3.45095442585563E-15,0.484752338922459));
#130325=DIRECTION('',(-0.529924709392052,5.88254176989232E-15,-0.848044693619239));
#130326=DIRECTION('',(1.,0.,0.));
#130327=DIRECTION('',(-0.529924185123396,-5.88254404234737E-15,0.84804502122311));
#130328=DIRECTION('center_axis',(-5.53239299512741E-17,-1.,-7.21882753539534E-15));
#130329=DIRECTION('ref_axis',(0.874649580953124,3.45097890568783E-15,-0.484755722543349));
#130330=DIRECTION('',(-1.,9.83319205199467E-31,-1.40816906889911E-16));
#130331=DIRECTION('',(-0.500005012714979,6.05598756357692E-15,-0.866022509672753));
#130332=DIRECTION('center_axis',(9.46835262113691E-7,0.999999999998207,
-1.63998885887388E-6));
#130333=DIRECTION('ref_axis',(0.866072335962825,-1.66725164348147E-10,0.499918702270574));
#130334=DIRECTION('',(-1.,9.83319205199467E-31,-1.40816906889911E-16));
#130335=DIRECTION('center_axis',(-9.46924648784811E-7,0.999999999998207,
-1.64014403517076E-6));
#130336=DIRECTION('ref_axis',(0.866043284546741,5.65134626076186E-11,-0.499969028332249));
#130337=DIRECTION('',(-0.500005169296822,-6.05598693139308E-15,0.866022419268956));
#130338=DIRECTION('',(-1.,9.83319205199467E-31,-1.40816906889911E-16));
#130339=DIRECTION('center_axis',(0.,-1.,-6.98296267768627E-15));
#130340=DIRECTION('ref_axis',(0.,6.98296267768627E-15,-1.));
#130341=DIRECTION('center_axis',(2.5057754547737E-16,1.,7.42579288178415E-15));
#130342=DIRECTION('ref_axis',(0.874649580936334,3.38052804894766E-15,-0.484755722573643));
#130343=DIRECTION('',(0.529924185123401,5.93414530587678E-15,-0.848045021223107));
#130344=DIRECTION('',(-1.,0.,0.));
#130345=DIRECTION('',(0.529924709392047,-5.93414301348781E-15,0.848044693619242));
#130346=DIRECTION('center_axis',(-2.50576144038582E-16,1.,7.42579081637246E-15));
#130347=DIRECTION('ref_axis',(0.874651456263127,-3.38050267703688E-15,0.484752338887387));
#130348=DIRECTION('',(1.,-9.83319205199467E-31,1.40816906889911E-16));
#130349=DIRECTION('',(0.500005169296811,5.91835086477038E-15,-0.866022419268963));
#130350=DIRECTION('center_axis',(-9.4705535579882E-7,-0.999999999998206,
-1.64037044329868E-6));
#130351=DIRECTION('ref_axis',(0.866072438648831,-1.66970090552065E-10,-0.499918524374589));
#130352=DIRECTION('',(1.,-9.83319205199467E-31,1.40816906889911E-16));
#130353=DIRECTION('center_axis',(9.46713286859869E-7,-0.999999999998207,
-1.63977760307947E-6));
#130354=DIRECTION('ref_axis',(0.8660431783397,5.62673641619407E-11,0.499969212303389));
#130355=DIRECTION('',(0.500005012714967,-5.9183514825864E-15,0.86602250967276));
#130356=DIRECTION('',(1.,-9.83319205199467E-31,1.40816906889911E-16));
#130357=DIRECTION('center_axis',(1.,0.,0.));
#130358=DIRECTION('ref_axis',(0.,-6.97886326506453E-15,1.));
#130359=DIRECTION('center_axis',(-1.,0.,0.));
#130360=DIRECTION('ref_axis',(0.,6.97886326506453E-15,-1.));
#130361=DIRECTION('center_axis',(-0.500005014362137,6.20016534342884E-15,
-0.866022508721753));
#130362=DIRECTION('ref_axis',(9.79094323195944E-13,-1.,-5.63853427197664E-13));
#130363=DIRECTION('center_axis',(-0.86601822301453,3.004221614602E-5,-0.500012436349559));
#130364=DIRECTION('ref_axis',(0.500012217441046,0.000989701298603201,-0.866017784402277));
#130365=DIRECTION('center_axis',(0.500005023014372,1.39506795850222E-14,
0.866022503726316));
#130366=DIRECTION('ref_axis',(-0.866022503726316,-3.41480999208039E-15,
0.500005023014372));
#130367=DIRECTION('center_axis',(1.,0.,0.));
#130368=DIRECTION('ref_axis',(0.,-6.82961998416066E-15,1.));
#130369=DIRECTION('center_axis',(-1.,9.83319205199467E-31,-1.4081690688991E-16));
#130370=DIRECTION('ref_axis',(1.4081690688991E-16,6.82961998416066E-15,
-1.));
#130371=DIRECTION('center_axis',(-1.,0.,0.));
#130372=DIRECTION('ref_axis',(0.,6.82961998416066E-15,-1.));
#130373=DIRECTION('center_axis',(-1.,9.83319205199467E-31,-1.4081690688991E-16));
#130374=DIRECTION('ref_axis',(1.4081690688991E-16,6.82961998416066E-15,
-1.));
#130375=DIRECTION('center_axis',(1.,0.,0.));
#130376=DIRECTION('ref_axis',(0.,-6.82961998416066E-15,1.));
#130377=DIRECTION('center_axis',(-0.529924213265765,-5.92186660939952E-15,
0.848045003637578));
#130378=DIRECTION('ref_axis',(-0.848045003637578,3.84166124109038E-15,-0.529924213265765));
#130379=DIRECTION('center_axis',(0.500005158533463,6.04740227518902E-15,
-0.866022425483271));
#130380=DIRECTION('ref_axis',(0.866022425483271,-3.41480999208032E-15,0.500005158533463));
#130381=DIRECTION('center_axis',(0.529924185004323,2.16250629064169E-8,
-0.848045021297516));
#130382=DIRECTION('ref_axis',(0.848037146343375,0.00430950302668586,0.529919264233193));
#130383=DIRECTION('center_axis',(-0.529924157141051,-5.92186685429947E-15,
0.848045038708645));
#130384=DIRECTION('ref_axis',(-0.848045038708645,3.84166124109037E-15,-0.529924157141051));
#130385=DIRECTION('center_axis',(0.500005172385372,1.05114548020227E-8,
-0.866022417485757));
#130386=DIRECTION('ref_axis',(0.866013458679463,0.00454855867658242,0.5));
#130387=DIRECTION('center_axis',(0.866037336481667,-3.44576747032758E-5,
-0.499979330205167));
#130388=DIRECTION('ref_axis',(0.499979069431688,-0.000963977562132558,0.866036951219452));
#130389=DIRECTION('center_axis',(-0.00024249581833115,0.999999970597889,
6.99630157351179E-15));
#130390=DIRECTION('ref_axis',(0.999999970597889,0.00024249581833115,9.21890050058242E-32));
#130391=DIRECTION('center_axis',(-1.,9.83319205199467E-31,-1.4081690688991E-16));
#130392=DIRECTION('ref_axis',(1.4081690688991E-16,6.82961998416066E-15,
-1.));
#130393=DIRECTION('center_axis',(1.,0.,0.));
#130394=DIRECTION('ref_axis',(0.,-6.82961998416066E-15,1.));
#130395=DIRECTION('center_axis',(0.,-6.98296267768627E-15,1.));
#130396=DIRECTION('ref_axis',(1.,1.22464679914735E-16,0.));
#130397=DIRECTION('center_axis',(0.000242495818331158,0.999999970597889,
6.98296247237242E-15));
#130398=DIRECTION('ref_axis',(0.999999970597889,-0.000242495818331158,-5.20911529687998E-32));
#130399=DIRECTION('center_axis',(0.529924676825566,1.14592471176548E-14,
0.848044713969328));
#130400=DIRECTION('ref_axis',(-0.848044713969328,-3.84166124109036E-15,
0.529924676825566));
#130401=DIRECTION('center_axis',(0.529924157141051,5.92186685429947E-15,
-0.848045038708645));
#130402=DIRECTION('ref_axis',(0.848045038708645,-3.84166124109037E-15,0.529924157141051));
#130403=DIRECTION('center_axis',(0.529924709439994,-2.52126420968272E-8,
0.848044693589281));
#130404=DIRECTION('ref_axis',(-0.848035979777037,-0.00453325469613692,0.529919264233204));
#130405=DIRECTION('center_axis',(0.529924742154432,-3.48753411745471E-14,
0.848044673146739));
#130406=DIRECTION('ref_axis',(-0.848044673146739,-3.84166124109014E-15,
0.529924742154432));
#130407=DIRECTION('center_axis',(-0.529924185162661,-2.16945438508739E-8,
0.848045021198574));
#130408=DIRECTION('ref_axis',(0.848037146343336,-0.00430950303668575,0.529919264233174));
#130409=DIRECTION('center_axis',(0.52992421326579,5.92186660939942E-15,
-0.848045003637563));
#130410=DIRECTION('ref_axis',(0.848045003637563,-3.84166124109038E-15,0.52992421326579));
#130411=DIRECTION('center_axis',(-0.000258180127964207,0.99999996667151,
6.95551716657602E-15));
#130412=DIRECTION('ref_axis',(0.99999996667151,0.000258180127964207,-1.33844997483071E-32));
#130413=DIRECTION('center_axis',(1.,0.,0.));
#130414=DIRECTION('ref_axis',(0.,-6.82961998416066E-15,1.));
#130415=DIRECTION('center_axis',(0.,-6.98296267768627E-15,1.));
#130416=DIRECTION('ref_axis',(1.,1.22464679914735E-16,0.));
#130417=DIRECTION('center_axis',(0.000258180127964191,0.99999996667151,
6.98372952115933E-15));
#130418=DIRECTION('ref_axis',(0.99999996667151,-0.000258180127964191,3.65206484909203E-32));
#130419=DIRECTION('center_axis',(1.,-9.83319205199467E-31,1.4081690688991E-16));
#130420=DIRECTION('ref_axis',(-1.4081690688991E-16,-6.82961998416066E-15,
1.));
#130421=DIRECTION('center_axis',(0.866018223015094,3.00422153149717E-5,
0.500012436348582));
#130422=DIRECTION('ref_axis',(0.500012217440065,-0.000989701305507211,-0.866017784402835));
#130423=DIRECTION('center_axis',(-0.529924742154432,-2.30316125713584E-14,
-0.848044673146739));
#130424=DIRECTION('ref_axis',(0.848044673146739,3.8416612410906E-15,-0.529924742154432));
#130425=DIRECTION('center_axis',(-0.50000500959944,1.0113261475945E-8,-0.866022511471535));
#130426=DIRECTION('ref_axis',(-0.866013834616175,0.0044764107713436,0.499999999999996));
#130427=DIRECTION('center_axis',(0.50000502301429,-6.04740282155761E-15,
0.866022503726363));
#130428=DIRECTION('ref_axis',(-0.866022503726363,-3.41480999208032E-15,
0.50000502301429));
#130429=DIRECTION('center_axis',(-0.529924709245859,2.52852559485652E-8,
-0.848044693710592));
#130430=DIRECTION('ref_axis',(-0.848035979777086,0.00453325468302945,0.529919264233239));
#130431=DIRECTION('center_axis',(-0.529924676825566,5.92186458665694E-15,
-0.848044713969328));
#130432=DIRECTION('ref_axis',(0.848044713969328,3.84166124109038E-15,-0.529924676825566));
#130433=DIRECTION('center_axis',(1.,0.,0.));
#130434=DIRECTION('ref_axis',(0.,-6.82961998416066E-15,1.));
#130435=DIRECTION('center_axis',(-1.,0.,0.));
#130436=DIRECTION('ref_axis',(0.,6.82961998416066E-15,-1.));
#130437=DIRECTION('center_axis',(1.,-9.83319205199467E-31,1.4081690688991E-16));
#130438=DIRECTION('ref_axis',(-1.4081690688991E-16,-6.82961998416066E-15,
1.));
#130439=DIRECTION('center_axis',(1.,-3.81527851617387E-28,5.46369598732844E-14));
#130440=DIRECTION('ref_axis',(-5.46369598732844E-14,-6.82961998416066E-15,
1.));
#130441=DIRECTION('center_axis',(1.,-9.83319205199467E-31,1.4081690688991E-16));
#130442=DIRECTION('ref_axis',(-1.4081690688991E-16,-6.82961998416066E-15,
1.));
#130443=DIRECTION('center_axis',(-0.866037336481684,-3.44576748086449E-5,
0.499979330205139));
#130444=DIRECTION('ref_axis',(0.499979069431657,0.000963977566348111,0.866036951219465));
#130445=DIRECTION('center_axis',(0.500005158533422,6.04740227518918E-15,
-0.866022425483294));
#130446=DIRECTION('ref_axis',(0.866022425483294,-3.41480999208032E-15,0.500005158533422));
#130447=DIRECTION('center_axis',(0.500005167509865,6.31729921158743E-15,
-0.866022420300671));
#130448=DIRECTION('ref_axis',(-5.94450122015092E-12,1.,-3.41808820158678E-12));
#130449=DIRECTION('center_axis',(-7.71409749859041E-19,-6.96824330280696E-15,
1.));
#130450=DIRECTION('ref_axis',(0.,-1.,-6.96824330280696E-15));
#130451=DIRECTION('',(0.994521895368273,0.104528463267654,7.29146948004066E-16));
#130452=DIRECTION('center_axis',(7.71409749859041E-19,6.96824330280696E-15,
-1.));
#130453=DIRECTION('ref_axis',(-1.08459293348099E-36,-1.,-6.96824330280696E-15));
#130454=DIRECTION('',(-0.994521895368273,-0.104528463267654,-7.29146948004066E-16));
#130455=DIRECTION('center_axis',(-7.71409749859041E-19,-6.96824330280696E-15,
1.));
#130456=DIRECTION('ref_axis',(2.55974201233206E-36,-1.,-6.96824330280696E-15));
#130457=DIRECTION('center_axis',(0.104528463267654,-0.994521895368273,-6.92998990261915E-15));
#130458=DIRECTION('ref_axis',(7.71409749859066E-19,6.96824330280696E-15,
-1.));
#130459=DIRECTION('center_axis',(0.104528463267637,-0.994521895368275,1.90905987588518E-14));
#130460=DIRECTION('ref_axis',(0.869860024050105,0.0914259726159642,0.48475233892244));
#130461=DIRECTION('',(-0.527021726387053,-0.0553922155203021,-0.848044693619247));
#130462=DIRECTION('',(0.994521895368273,0.104528463267654,7.29146948004067E-16));
#130463=DIRECTION('',(-0.527021204990394,-0.0553921607193182,0.848045021223118));
#130464=DIRECTION('center_axis',(0.10452846326765,-0.994521895368274,-1.18885524848236E-14));
#130465=DIRECTION('ref_axis',(0.869858159031309,0.0914257765945981,-0.48475572254563));
#130466=DIRECTION('',(-0.994521895368273,-0.104528463267654,-8.69963854893977E-16));
#130467=DIRECTION('',(-0.497265932938934,-0.05226475560521,-0.866022509672756));
#130468=DIRECTION('center_axis',(-0.104527521619063,0.994521994337725,-1.63998885964307E-6));
#130469=DIRECTION('ref_axis',(0.861327901105178,0.0905292101910039,0.499918702270621));
#130470=DIRECTION('',(-0.994521895368273,-0.104528463267654,-8.69963854893977E-16));
#130471=DIRECTION('center_axis',(-0.104529405004769,0.994521796385911,-1.6401440381083E-6));
#130472=DIRECTION('ref_axis',(0.861299008814395,0.0905261737133511,-0.499969028328917));
#130473=DIRECTION('',(-0.497266088663003,-0.0522647719724915,0.86602241926896));
#130474=DIRECTION('',(-0.994521895368273,-0.104528463267654,-8.69963854893977E-16));
#130475=DIRECTION('center_axis',(0.104528463267654,-0.994521895368273,-6.92998990261915E-15));
#130476=DIRECTION('ref_axis',(7.71409749859066E-19,6.96824330280696E-15,
-1.));
#130477=DIRECTION('center_axis',(-0.104528463267662,0.994521895368273,-4.47974441404753E-15));
#130478=DIRECTION('ref_axis',(0.869858159016179,0.0914257765930096,-0.484755722573081));
#130479=DIRECTION('',(0.527021204990417,0.0553921607193179,-0.848045021223103));
#130480=DIRECTION('',(-0.994521895368273,-0.104528463267654,-7.29146948004067E-16));
#130481=DIRECTION('',(0.527021726387063,0.0553922155203017,0.848044693619241));
#130482=DIRECTION('center_axis',(-0.104528463267657,0.994521895368273,1.39216640785751E-14));
#130483=DIRECTION('ref_axis',(0.869860024068681,0.0914259726179182,0.484752338888738));
#130484=DIRECTION('',(0.994521895368273,0.104528463267654,8.69963854893977E-16));
#130485=DIRECTION('',(0.497266088663018,0.052264771972485,-0.866022419268951));
#130486=DIRECTION('center_axis',(0.104527521400192,-0.994521994360729,-1.64037041421999E-6));
#130487=DIRECTION('ref_axis',(0.861328003227311,0.0905292209242257,-0.49991852437703));
#130488=DIRECTION('',(0.994521895368273,0.104528463267654,8.69963854893977E-16));
#130489=DIRECTION('center_axis',(0.10452940479455,-0.994521796408007,-1.63977758816116E-6));
#130490=DIRECTION('ref_axis',(0.861298903188812,0.0905261626114036,0.49996921230072));
#130491=DIRECTION('',(0.497265932938937,0.0522647556052066,0.866022509672755));
#130492=DIRECTION('',(0.994521895368273,0.104528463267654,8.69963854893977E-16));
#130493=DIRECTION('center_axis',(-3.07718727278886E-18,-6.95368519647906E-15,
1.));
#130494=DIRECTION('ref_axis',(0.,-1.,-6.95368519647906E-15));
#130495=DIRECTION('',(0.978147600733805,0.20791169081776,1.44876238996227E-15));
#130496=DIRECTION('center_axis',(3.07718727278886E-18,6.95368519647906E-15,
-1.));
#130497=DIRECTION('ref_axis',(2.06146211212399E-12,-1.,-6.95368519647905E-15));
#130498=DIRECTION('',(-0.978147600733805,-0.20791169081776,-1.44876238996227E-15));
#130499=DIRECTION('center_axis',(-3.07718727278886E-18,-6.95368519647906E-15,
1.));
#130500=DIRECTION('ref_axis',(1.06288922528842E-35,-1.,-6.95368519647906E-15));
#130501=DIRECTION('center_axis',(0.20791169081776,-0.978147600733806,-6.80109070798532E-15));
#130502=DIRECTION('ref_axis',(3.07718727278892E-18,6.95368519647906E-15,
-1.));
#130503=DIRECTION('center_axis',(0.207911690817738,-0.97814760073381,3.2805505448422E-14));
#130504=DIRECTION('ref_axis',(0.855538223403851,0.181850263143999,0.484752338921063));
#130505=DIRECTION('',(-0.518344583061401,-0.110177542335806,-0.848044693619236));
#130506=DIRECTION('',(0.978147600733806,0.20791169081776,1.44876238996227E-15));
#130507=DIRECTION('',(-0.518344070249267,-0.110177433334231,0.848045021223109));
#130508=DIRECTION('center_axis',(0.207911690817745,-0.978147600733809,-5.5135315871643E-14));
#130509=DIRECTION('ref_axis',(0.855536389092617,0.181849873249127,-0.48475572254244));
#130510=DIRECTION('',(-0.978147600733806,-0.20791169081776,-1.58957929685218E-15));
#130511=DIRECTION('',(-0.489078703542047,-0.103956887610915,-0.866022509672747));
#130512=DIRECTION('center_axis',(-0.207910764672755,0.97814779759017,-1.63998884845435E-6));
#130513=DIRECTION('ref_axis',(0.847146577517719,0.180066563577246,0.499918702272176));
#130514=DIRECTION('',(-0.978147600733806,-0.20791169081776,-1.58957929685218E-15));
#130515=DIRECTION('center_axis',(-0.207912617049438,0.978147403855351,-1.64014399912025E-6));
#130516=DIRECTION('ref_axis',(0.847118160900897,0.180060523667102,-0.499969028329366));
#130517=DIRECTION('',(-0.489078856702207,-0.10395692016612,0.866022419268945));
#130518=DIRECTION('',(-0.978147600733806,-0.20791169081776,-1.58957929685218E-15));
#130519=DIRECTION('center_axis',(0.20791169081776,-0.978147600733806,-6.80109070798532E-15));
#130520=DIRECTION('ref_axis',(3.07718727278892E-18,6.95368519647906E-15,
-1.));
#130521=DIRECTION('center_axis',(-0.207911690817755,0.978147600733807,2.12270966081019E-14));
#130522=DIRECTION('ref_axis',(0.855536389075087,0.181849873245393,-0.484755722574778));
#130523=DIRECTION('',(0.518344070249257,0.110177433334232,-0.848045021223115));
#130524=DIRECTION('',(-0.978147600733806,-0.20791169081776,-1.44876238996227E-15));
#130525=DIRECTION('',(0.518344583061396,0.110177542335808,0.848044693619239));
#130526=DIRECTION('center_axis',(-0.207911690817758,0.978147600733806,-5.58244945724969E-15));
#130527=DIRECTION('ref_axis',(0.855538223421779,0.181850263147814,0.48475233888799));
#130528=DIRECTION('',(0.978147600733806,0.20791169081776,1.58957929685218E-15));
#130529=DIRECTION('',(0.489078856702179,0.10395692016613,-0.86602241926896));
#130530=DIRECTION('center_axis',(0.207910764457463,-0.978147797635931,-1.64037042063166E-6));
#130531=DIRECTION('ref_axis',(0.847146677960003,0.180066584926648,-0.499918524375908));
#130532=DIRECTION('',(0.978147600733806,0.20791169081776,1.58957929685218E-15));
#130533=DIRECTION('center_axis',(0.207912616842675,-0.978147403899301,-1.63977751440231E-6));
#130534=DIRECTION('ref_axis',(0.847118057016758,0.180060501585604,0.499969212297011));
#130535=DIRECTION('',(0.489078703542037,0.103956887610914,0.866022509672752));
#130536=DIRECTION('',(0.978147600733806,0.20791169081776,1.58957929685218E-15));
#130537=DIRECTION('center_axis',(-6.89206998773325E-18,-6.93944786036197E-15,
1.));
#130538=DIRECTION('ref_axis',(0.,-1.,-6.93944786036197E-15));
#130539=DIRECTION('',(0.951056516295153,0.309016994374948,2.15096206850332E-15));
#130540=DIRECTION('center_axis',(6.89206998773325E-18,6.93944786036197E-15,
-1.));
#130541=DIRECTION('ref_axis',(-6.04138961080025E-12,-1.,-6.93944786036201E-15));
#130542=DIRECTION('',(-0.951056516295153,-0.309016994374948,-2.15096206850332E-15));
#130543=DIRECTION('center_axis',(-6.89206998773325E-18,-6.93944786036197E-15,
1.));
#130544=DIRECTION('ref_axis',(-2.36830503925458E-35,-1.,-6.93944786036197E-15));
#130545=DIRECTION('center_axis',(0.309016994374948,-0.951056516295153,-6.59767734033508E-15));
#130546=DIRECTION('ref_axis',(6.89206998773322E-18,6.93944786036197E-15,
-1.));
#130547=DIRECTION('center_axis',(0.309016994374975,-0.951056516295145,-5.00352877217599E-14));
#130548=DIRECTION('ref_axis',(0.831842966947628,0.270282164134104,0.484752338922417));
#130549=DIRECTION('',(-0.503988348013119,-0.163755740941345,-0.848044693619245));
#130550=DIRECTION('',(0.951056516295153,0.309016994374948,2.15096206850332E-15));
#130551=DIRECTION('',(-0.503987849403997,-0.163755578933432,0.848045021223113));
#130552=DIRECTION('center_axis',(0.309016994374943,-0.951056516295155,-1.8608169106679E-14));
#130553=DIRECTION('ref_axis',(0.831841183440077,0.270281584637376,-0.484755722543759));
#130554=DIRECTION('',(-0.951056516295153,-0.309016994374948,-2.29177897539323E-15));
#130555=DIRECTION('',(-0.47553302552285,-0.154510046201597,-0.866022509672736));
#130556=DIRECTION('center_axis',(-0.30901609388053,0.951056808881641,-1.63998886386027E-6));
#130557=DIRECTION('ref_axis',(0.823683738752015,0.26763107001197,0.499918702270429));
#130558=DIRECTION('',(-0.951056516295153,-0.309016994374948,-2.29177897539323E-15));
#130559=DIRECTION('center_axis',(-0.30901789495323,0.951056223677646,-1.64014403819393E-6));
#130560=DIRECTION('ref_axis',(0.823656109144305,0.267622092842945,-0.499969028332382));
#130561=DIRECTION('',(-0.475533174441002,-0.154510094588054,0.866022419268955));
#130562=DIRECTION('',(-0.951056516295153,-0.309016994374948,-2.29177897539323E-15));
#130563=DIRECTION('center_axis',(0.309016994374948,-0.951056516295153,-6.59767734033508E-15));
#130564=DIRECTION('ref_axis',(6.89206998773322E-18,6.93944786036197E-15,
-1.));
#130565=DIRECTION('center_axis',(-0.309016994374928,0.95105651629516,3.79055296573235E-14));
#130566=DIRECTION('ref_axis',(0.831841183424877,0.270281584632433,-0.484755722572598));
#130567=DIRECTION('',(0.503987849404017,0.163755578933437,-0.848045021223101));
#130568=DIRECTION('',(-0.951056516295153,-0.309016994374948,-2.15096206850332E-15));
#130569=DIRECTION('',(0.503988348013119,0.163755740941342,0.848044693619245));
#130570=DIRECTION('center_axis',(-0.309016994374936,0.951056516295157,-1.18540902055188E-14));
#130571=DIRECTION('ref_axis',(0.831842966965641,0.27028216413995,0.484752338888245));
#130572=DIRECTION('',(0.951056516295153,0.309016994374948,2.29177897539323E-15));
#130573=DIRECTION('',(0.475533174441018,0.154510094588057,-0.866022419268946));
#130574=DIRECTION('center_axis',(0.309016093671233,-0.951056808949645,-1.64037046624666E-6));
#130575=DIRECTION('ref_axis',(0.823683836411332,0.267631101743181,-0.499918524376164));
#130576=DIRECTION('',(0.951056516295153,0.309016994374948,2.29177897539323E-15));
#130577=DIRECTION('center_axis',(0.309017894752258,-0.951056223742947,-1.639777670527E-6));
#130578=DIRECTION('ref_axis',(0.823656008138232,0.267622060023833,0.49996921229851));
#130579=DIRECTION('',(0.475533025522778,0.154510046201593,0.866022509672777));
#130580=DIRECTION('',(0.951056516295153,0.309016994374948,2.29177897539323E-15));
#130581=DIRECTION('center_axis',(-1.21742612413517E-17,-6.92568728168955E-15,
1.));
#130582=DIRECTION('ref_axis',(0.,-1.,-6.92568728168955E-15));
#130583=DIRECTION('',(0.913545457642601,0.406736643075801,2.82805253700437E-15));
#130584=DIRECTION('center_axis',(1.21742612413517E-17,6.92568728168955E-15,
-1.));
#130585=DIRECTION('ref_axis',(-3.11436113529516E-35,-1.,-6.92568728168955E-15));
#130586=DIRECTION('',(-0.913545457642601,-0.406736643075801,-2.82805253700437E-15));
#130587=DIRECTION('center_axis',(-1.21742612413517E-17,-6.92568728168955E-15,
1.));
#130588=DIRECTION('ref_axis',(-3.04711942787957E-35,-1.,-6.92568728168955E-15));
#130589=DIRECTION('center_axis',(0.406736643075801,-0.913545457642601,-6.32197843909138E-15));
#130590=DIRECTION('ref_axis',(1.21742612413516E-17,6.92568728168955E-15,
-1.));
#130591=DIRECTION('center_axis',(0.406736643075802,-0.9135454576426,1.92973561461327E-15));
#130592=DIRECTION('ref_axis',(0.799033864871343,0.355752797173669,0.484752338923573));
#130593=DIRECTION('',(-0.484110311157683,-0.21553979738103,-0.848044693619243));
#130594=DIRECTION('',(0.913545457642601,0.406736643075801,2.82805253700437E-15));
#130595=DIRECTION('',(-0.484109832214428,-0.215539584141767,0.848045021223115));
#130596=DIRECTION('center_axis',(0.406736643075783,-0.913545457642609,-5.80299199549056E-14));
#130597=DIRECTION('ref_axis',(0.799032151707775,0.355752034424116,-0.484755722545228));
#130598=DIRECTION('',(-0.913545457642601,-0.406736643075801,-2.96886944389428E-15));
#130599=DIRECTION('',(-0.456777308164342,-0.20337036039276,-0.866022509672732));
#130600=DIRECTION('center_axis',(-0.40673577809802,0.913545842753558,-1.63998889148739E-6));
#130601=DIRECTION('ref_axis',(0.791196448577878,0.352263354438628,0.499918702268077));
#130602=DIRECTION('',(-0.913545457642601,-0.406736643075801,-2.96886944389428E-15));
#130603=DIRECTION('center_axis',(-0.406737508133751,0.913545072492024,-1.6401440001529E-6));
#130604=DIRECTION('ref_axis',(0.791169908694268,0.352251538365472,-0.499969028336619));
#130605=DIRECTION('',(-0.45677745120893,-0.203370424080359,0.866022419268952));
#130606=DIRECTION('',(-0.913545457642601,-0.406736643075801,-2.96886944389428E-15));
#130607=DIRECTION('center_axis',(0.406736643075801,-0.913545457642601,-6.32197843909138E-15));
#130608=DIRECTION('ref_axis',(1.21742612413516E-17,6.92568728168955E-15,
-1.));
#130609=DIRECTION('center_axis',(-0.406736643075821,0.913545457642592,-5.01731374373314E-14));
#130610=DIRECTION('ref_axis',(0.799032151693526,0.355752034417755,-0.484755722573383));
#130611=DIRECTION('',(0.484109832214453,0.215539584141773,-0.848045021223098));
#130612=DIRECTION('',(-0.913545457642601,-0.406736643075801,-2.82805253700437E-15));
#130613=DIRECTION('',(0.484110311157685,0.215539797381037,0.84804469361924));
#130614=DIRECTION('center_axis',(-0.406736643075817,0.913545457642593,4.39704043669841E-14));
#130615=DIRECTION('ref_axis',(0.799033864889297,0.355752797181655,0.484752338888119));
#130616=DIRECTION('',(0.9135454576426,0.406736643075801,2.96886944389428E-15));
#130617=DIRECTION('',(0.45677745120893,0.203370424080376,-0.866022419268948));
#130618=DIRECTION('center_axis',(0.406735777896989,-0.913545842843062,-1.64037036589386E-6));
#130619=DIRECTION('ref_axis',(0.791196542384911,0.352263396203918,-0.499918524374765));
#130620=DIRECTION('',(0.913545457642601,0.406736643075801,2.96886944389428E-15));
#130621=DIRECTION('center_axis',(0.406737507940689,-0.913545072577981,-1.63977759702633E-6));
#130622=DIRECTION('ref_axis',(0.791169811673513,0.352251495168791,0.499969212299967));
#130623=DIRECTION('',(0.45677730816427,0.203370360392743,0.866022509672774));
#130624=DIRECTION('',(0.913545457642601,0.406736643075801,2.96886944389428E-15));
#130625=DIRECTION('center_axis',(-1.88658882409001E-17,-6.91255422424131E-15,
1.));
#130626=DIRECTION('ref_axis',(0.,-1.,-6.91255422424131E-15));
#130627=DIRECTION('',(0.866025403784438,0.500000000000001,3.47261545060224E-15));
#130628=DIRECTION('center_axis',(1.88658882409001E-17,6.91255422424131E-15,
-1.));
#130629=DIRECTION('ref_axis',(3.83604259468484E-12,-1.,-6.91255422424124E-15));
#130630=DIRECTION('',(-0.866025403784438,-0.500000000000001,-3.47261545060224E-15));
#130631=DIRECTION('center_axis',(-1.88658882409001E-17,-6.91255422424131E-15,
1.));
#130632=DIRECTION('ref_axis',(-1.77724617242827E-35,-1.,-6.91255422424131E-15));
#130633=DIRECTION('center_axis',(0.500000000000001,-0.866025403784438,-5.97701461910995E-15));
#130634=DIRECTION('ref_axis',(1.88658882408999E-17,6.91255422424131E-15,
-1.));
#130635=DIRECTION('center_axis',(0.500000000000029,-0.866025403784422,-5.32055676600525E-14));
#130636=DIRECTION('ref_axis',(0.757470380563957,0.437325728121773,0.484752338922729));
#130637=DIRECTION('',(-0.458928260426595,-0.264962354696009,-0.848044693619249));
#130638=DIRECTION('',(0.866025403784438,0.500000000000001,3.47261545060224E-15));
#130639=DIRECTION('',(-0.458927806396613,-0.264962092561708,0.848045021223115));
#130640=DIRECTION('center_axis',(0.500000000000022,-0.866025403784426,2.06757434518667E-14));
#130641=DIRECTION('ref_axis',(0.757468756514555,0.437324790476423,-0.484755722543887));
#130642=DIRECTION('',(-0.866025403784438,-0.500000000000001,-3.61343235749215E-15));
#130643=DIRECTION('',(-0.433017043030787,-0.250002506357499,-0.866022509672723));
#130644=DIRECTION('center_axis',(-0.499999180015709,0.86602587720052,-1.63998889217594E-6));
#130645=DIRECTION('ref_axis',(0.750040644542496,0.433036167837267,0.499918702269771));
#130646=DIRECTION('',(-0.866025403784438,-0.500000000000001,-3.61343235749215E-15));
#130647=DIRECTION('center_axis',(-0.500000820059939,0.866024930320542,-1.64014409121096E-6));
#130648=DIRECTION('ref_axis',(0.750015485167105,0.433021642322879,-0.499969028330305));
#130649=DIRECTION('',(-0.433017178634592,-0.25000258464845,0.866022419268943));
#130650=DIRECTION('',(-0.866025403784438,-0.500000000000001,-3.61343235749215E-15));
#130651=DIRECTION('center_axis',(0.500000000000001,-0.866025403784438,-5.97701461910995E-15));
#130652=DIRECTION('ref_axis',(1.88658882408999E-17,6.91255422424131E-15,
-1.));
#130653=DIRECTION('center_axis',(-0.499999999999999,0.866025403784439,1.32324758076477E-14));
#130654=DIRECTION('ref_axis',(0.757468756499566,0.437324790467762,-0.484755722575123));
#130655=DIRECTION('',(0.458927806396622,0.264962092561705,-0.848045021223111));
#130656=DIRECTION('',(-0.866025403784438,-0.500000000000001,-3.47261545060224E-15));
#130657=DIRECTION('',(0.458928260426604,0.26496235469602,0.848044693619241));
#130658=DIRECTION('center_axis',(-0.500000000000014,0.866025403784431,3.62514619075765E-14));
#130659=DIRECTION('ref_axis',(0.75747038058095,0.437325728131575,0.484752338887332));
#130660=DIRECTION('',(0.866025403784438,0.500000000000001,3.61343235749215E-15));
#130661=DIRECTION('',(0.433017178634604,0.25000258464844,-0.866022419268939));
#130662=DIRECTION('center_axis',(0.499999179825138,-0.866025877310545,-1.64037034781974E-6));
#130663=DIRECTION('ref_axis',(0.750040733469403,0.433036219178925,-0.499918524377625));
#130664=DIRECTION('',(0.866025403784438,0.500000000000001,3.61343235749215E-15));
#130665=DIRECTION('center_axis',(0.500000819876823,-0.866024930426264,-1.63977751905006E-6));
#130666=DIRECTION('ref_axis',(0.750015393191207,0.433021589220285,0.499969212297495));
#130667=DIRECTION('',(0.433017043030726,0.250002506357484,0.866022509672758));
#130668=DIRECTION('',(0.866025403784438,0.500000000000001,3.61343235749215E-15));
#130669=DIRECTION('center_axis',(-2.68936361206584E-17,-6.90019257654293E-15,
1.));
#130670=DIRECTION('ref_axis',(0.,-1.,-6.90019257654294E-15));
#130671=DIRECTION('',(0.809016994374947,0.587785252292474,4.07758884313209E-15));
#130672=DIRECTION('center_axis',(2.68936361206584E-17,6.90019257654293E-15,
-1.));
#130673=DIRECTION('ref_axis',(-1.21098210448278E-35,-1.,-6.90019257654293E-15));
#130674=DIRECTION('',(-0.809016994374947,-0.587785252292474,-4.07758884313209E-15));
#130675=DIRECTION('center_axis',(-2.68936361206584E-17,-6.90019257654293E-15,
1.));
#130676=DIRECTION('ref_axis',(3.73887388675131E-35,-1.,-6.90019257654293E-15));
#130677=DIRECTION('center_axis',(0.587785252292474,-0.809016994374947,-5.56656537619084E-15));
#130678=DIRECTION('ref_axis',(2.6893636120658E-17,6.90019257654294E-15,
-1.));
#130679=DIRECTION('center_axis',(0.587785252292488,-0.809016994374937,-2.2605474342611E-14));
#130680=DIRECTION('ref_axis',(0.707607892256329,0.514107226876464,0.484752338921584));
#130681=DIRECTION('',(-0.428718095637387,-0.311481929006017,-0.848044693619235));
#130682=DIRECTION('',(0.809016994374947,0.587785252292474,4.07758884313209E-15));
#130683=DIRECTION('',(-0.428717671495138,-0.311481620848666,0.848045021223092));
#130684=DIRECTION('center_axis',(0.587785252292496,-0.809016994374931,6.42326429904636E-14));
#130685=DIRECTION('ref_axis',(0.707606375113785,0.514106124607871,-0.484755722543847));
#130686=DIRECTION('',(-0.809016994374947,-0.587785252292474,-4.21840575002201E-15));
#130687=DIRECTION('',(-0.404512552559103,-0.293895572546151,-0.86602250967275));
#130688=DIRECTION('center_axis',(-0.587784486285606,0.809017550909297,-1.63998889613513E-6));
#130689=DIRECTION('ref_axis',(0.700667238250726,0.509064546363162,0.499918702268848));
#130690=DIRECTION('',(-0.809016994374947,-0.587785252292474,-4.21840575002201E-15));
#130691=DIRECTION('center_axis',(-0.587786018369567,0.809016437785142,-1.6401440982681E-6));
#130692=DIRECTION('ref_axis',(0.700643735030324,0.509047470549884,-0.499969028330278));
#130693=DIRECTION('',(-0.404512679236431,-0.293895664582696,0.866022419268959));
#130694=DIRECTION('',(-0.809016994374947,-0.587785252292474,-4.21840575002201E-15));
#130695=DIRECTION('center_axis',(0.587785252292474,-0.809016994374947,-5.56656537619084E-15));
#130696=DIRECTION('ref_axis',(2.6893636120658E-17,6.90019257654294E-15,
-1.));
#130697=DIRECTION('center_axis',(-0.587785252292482,0.809016994374941,-9.09732711775792E-15));
#130698=DIRECTION('ref_axis',(0.707606375100825,0.514106124598469,-0.484755722572735));
#130699=DIRECTION('',(0.428717671495133,0.311481620848643,-0.848045021223103));
#130700=DIRECTION('',(-0.809016994374947,-0.587785252292474,-4.07758884313209E-15));
#130701=DIRECTION('',(0.428718095637375,0.311481929006018,0.848044693619241));
#130702=DIRECTION('center_axis',(-0.587785252292472,0.809016994374949,2.06757387305573E-15));
#130703=DIRECTION('ref_axis',(0.707607892271538,0.514107226887505,0.484752338887674));
#130704=DIRECTION('',(0.809016994374947,0.587785252292474,4.21840575002201E-15));
#130705=DIRECTION('',(0.404512679236465,0.293895664582661,-0.866022419268954));
#130706=DIRECTION('center_axis',(0.587784486107541,-0.809017551038668,-1.64037047777937E-6));
#130707=DIRECTION('ref_axis',(0.700667321324406,0.509064606719412,-0.499918524375414));
#130708=DIRECTION('',(0.809016994374947,0.587785252292474,4.21840575002201E-15));
#130709=DIRECTION('center_axis',(0.587786018198601,-0.809016437909357,-1.63977768550205E-6));
#130710=DIRECTION('ref_axis',(0.700643649108103,0.509047408123459,0.499969212299387));
#130711=DIRECTION('',(0.404512552559084,0.293895572546173,0.866022509672752));
#130712=DIRECTION('',(0.809016994374947,0.587785252292474,4.21840575002201E-15));
#130713=DIRECTION('center_axis',(-3.61695511949416E-17,-6.88873777539344E-15,
1.));
#130714=DIRECTION('ref_axis',(0.,-1.,-6.88873777539344E-15));
#130715=DIRECTION('',(0.743144825477393,0.669130606358859,4.63634449950655E-15));
#130716=DIRECTION('center_axis',(3.61695511949416E-17,6.88873777539344E-15,
-1.));
#130717=DIRECTION('ref_axis',(6.85846605685609E-35,-1.,-6.88873777539344E-15));
#130718=DIRECTION('',(-0.743144825477393,-0.669130606358859,-4.63634449950655E-15));
#130719=DIRECTION('center_axis',(-3.61695511949416E-17,-6.88873777539344E-15,
1.));
#130720=DIRECTION('ref_axis',(-9.8293973350875E-35,-1.,-6.88873777539344E-15));
#130721=DIRECTION('center_axis',(0.669130606358859,-0.743144825477393,-5.09512767813149E-15));
#130722=DIRECTION('ref_axis',(3.61695511949414E-17,6.88873777539344E-15,
-1.));
#130723=DIRECTION('center_axis',(0.669130606358863,-0.74314482547739,2.56379160227189E-14));
#130724=DIRECTION('ref_axis',(0.649992703803497,0.585256059268782,0.484752338923078));
#130725=DIRECTION('',(-0.393810805677315,-0.354588842120017,-0.848044693619251));
#130726=DIRECTION('',(0.743144825477393,0.669130606358859,4.63634449950655E-15));
#130727=DIRECTION('',(-0.393810416069769,-0.354588491315852,0.848045021223109));
#130728=DIRECTION('center_axis',(0.669130606358859,-0.743144825477393,4.41082526973097E-15));
#130729=DIRECTION('ref_axis',(0.649991310190666,0.585254804454127,-0.484755722544853));
#130730=DIRECTION('',(-0.743144825477393,-0.669130606358859,-4.77716140639646E-15));
#130731=DIRECTION('',(-0.3715761379119,-0.334568657340434,-0.866022509672754));
#130732=DIRECTION('center_axis',(-0.669129902721922,0.743145459032525,-1.63998885774954E-6));
#130733=DIRECTION('ref_axis',(0.643617175072105,0.579515507190106,0.499918702269076));
#130734=DIRECTION('',(-0.743144825477393,-0.669130606358859,-4.77716140639646E-15));
#130735=DIRECTION('center_axis',(-0.669131310059706,0.743144191859892,-1.64014388379194E-6));
#130736=DIRECTION('ref_axis',(0.64359558551269,0.579496068163846,-0.499969028331978));
#130737=DIRECTION('',(-0.371576254274913,-0.33456876211417,0.866022419268934));
#130738=DIRECTION('',(-0.743144825477393,-0.669130606358859,-4.77716140639646E-15));
#130739=DIRECTION('center_axis',(0.669130606358859,-0.743144825477393,-5.09512767813149E-15));
#130740=DIRECTION('ref_axis',(3.61695511949414E-17,6.88873777539344E-15,
-1.));
#130741=DIRECTION('center_axis',(-0.669130606358859,0.743144825477393,-3.225415978114E-14));
#130742=DIRECTION('ref_axis',(0.649991310179485,0.585254804444041,-0.484755722572022));
#130743=DIRECTION('',(0.393810416069769,0.354588491315851,-0.84804502122311));
#130744=DIRECTION('',(-0.743144825477393,-0.669130606358859,-4.63634449950655E-15));
#130745=DIRECTION('',(0.393810805677318,0.354588842120046,0.848044693619238));
#130746=DIRECTION('center_axis',(-0.669130606358895,0.743144825477361,1.30119315744295E-13));
#130747=DIRECTION('ref_axis',(0.649992703818358,0.585256059282112,0.484752338887059));
#130748=DIRECTION('',(0.743144825477393,0.669130606358859,4.77716140639646E-15));
#130749=DIRECTION('',(0.371576254274905,0.334568762114163,-0.86602241926894));
#130750=DIRECTION('center_axis',(0.66912990255837,-0.743145459179787,-1.64037045350906E-6));
#130751=DIRECTION('ref_axis',(0.643617251380043,0.579515575897775,-0.499918524379592));
#130752=DIRECTION('',(0.743144825477393,0.669130606358859,4.77716140639646E-15));
#130753=DIRECTION('center_axis',(0.669131309902701,-0.743144192001261,-1.63977754710756E-6));
#130754=DIRECTION('ref_axis',(0.643595506588125,0.579495997099558,0.499969212297282));
#130755=DIRECTION('',(0.371576137911895,0.334568657340433,0.866022509672757));
#130756=DIRECTION('',(0.743144825477393,0.669130606358859,4.77716140639646E-15));
#130757=DIRECTION('center_axis',(-4.6592004597086E-17,-6.8783153219913E-15,
1.));
#130758=DIRECTION('ref_axis',(0.,-1.,-6.8783153219913E-15));
#130759=DIRECTION('',(0.669130606358857,0.743144825477395,5.14276057582724E-15));
#130760=DIRECTION('center_axis',(4.6592004597086E-17,6.8783153219913E-15,
-1.));
#130761=DIRECTION('ref_axis',(3.5473846082823E-12,-1.,-6.87831532199113E-15));
#130762=DIRECTION('',(-0.669130606358857,-0.743144825477395,-5.14276057582724E-15));
#130763=DIRECTION('center_axis',(-4.6592004597086E-17,-6.8783153219913E-15,
1.));
#130764=DIRECTION('ref_axis',(7.23989575295994E-35,-1.,-6.8783153219913E-15));
#130765=DIRECTION('center_axis',(0.743144825477395,-0.669130606358857,-4.56786669500651E-15));
#130766=DIRECTION('ref_axis',(4.65920045970859E-17,6.8783153219913E-15,
-1.));
#130767=DIRECTION('center_axis',(0.743144825477392,-0.66913060635886,4.24541835214864E-14));
#130768=DIRECTION('ref_axis',(0.585256059269044,0.649992703803843,0.484752338922299));
#130769=DIRECTION('',(-0.354588842120053,-0.393810805677299,-0.848044693619244));
#130770=DIRECTION('',(0.669130606358857,0.743144825477395,5.14276057582724E-15));
#130771=DIRECTION('',(-0.354588491315835,-0.393810416069765,0.848045021223118));
#130772=DIRECTION('center_axis',(0.743144825477363,-0.669130606358893,-8.68381224978382E-14));
#130773=DIRECTION('ref_axis',(0.585254804454296,0.649991310190854,-0.484755722544398));
#130774=DIRECTION('',(-0.669130606358857,-0.743144825477395,-5.28357748271715E-15));
#130775=DIRECTION('',(-0.334568657340461,-0.371576137911926,-0.866022509672733));
#130776=DIRECTION('center_axis',(-0.743144191919596,0.669131309993398,-1.6399889042252E-6));
#130777=DIRECTION('ref_axis',(0.579515507436744,0.643617174847681,0.499918702272102));
#130778=DIRECTION('',(-0.669130606358857,-0.743144825477395,-5.28357748271715E-15));
#130779=DIRECTION('center_axis',(-0.743145459092377,0.669129902655449,-1.64014418399028E-6));
#130780=DIRECTION('ref_axis',(0.579496068079923,0.643595585588318,-0.499969028331896));
#130781=DIRECTION('',(-0.334568762114163,-0.371576254274904,0.86602241926894));
#130782=DIRECTION('',(-0.669130606358857,-0.743144825477395,-5.28357748271715E-15));
#130783=DIRECTION('center_axis',(0.743144825477395,-0.669130606358857,-4.56786669500651E-15));
#130784=DIRECTION('ref_axis',(4.65920045970859E-17,6.8783153219913E-15,
-1.));
#130785=DIRECTION('center_axis',(-0.743144825477411,0.66913060635884,-6.75407619348667E-14));
#130786=DIRECTION('ref_axis',(0.585254804443858,0.649991310179243,-0.484755722572568));
#130787=DIRECTION('',(0.354588491315848,0.393810416069791,-0.848045021223101));
#130788=DIRECTION('',(-0.669130606358857,-0.743144825477395,-5.14276057582724E-15));
#130789=DIRECTION('',(0.354588842120031,0.393810805677304,0.84804469361925));
#130790=DIRECTION('center_axis',(-0.743144825477382,0.669130606358872,-2.1227091763372E-14));
#130791=DIRECTION('ref_axis',(0.585256059281954,0.649992703818144,0.484752338887536));
#130792=DIRECTION('',(0.669130606358857,0.743144825477395,5.28357748271715E-15));
#130793=DIRECTION('',(0.334568762114167,0.371576254274874,-0.866022419268952));
#130794=DIRECTION('center_axis',(0.743144191772429,-0.669131310156843,-1.64037028413086E-6));
#130795=DIRECTION('ref_axis',(0.579515576147915,0.643617251158851,-0.499918524374397));
#130796=DIRECTION('',(0.669130606358857,0.743144825477395,5.28357748271715E-15));
#130797=DIRECTION('center_axis',(0.743145458950857,-0.669129902812624,-1.63977741490995E-6));
#130798=DIRECTION('ref_axis',(0.57949599701582,0.643595506663342,0.499969212297514));
#130799=DIRECTION('',(0.334568657340468,0.37157613791193,0.866022509672728));
#130800=DIRECTION('',(0.669130606358857,0.743144825477395,5.28357748271715E-15));
#130801=DIRECTION('center_axis',(-5.8046805746579E-17,-6.86903940691701E-15,
1.));
#130802=DIRECTION('ref_axis',(0.,-1.,-6.86903940691702E-15));
#130803=DIRECTION('',(0.587785252292471,0.809016994374949,5.59128867158761E-15));
#130804=DIRECTION('center_axis',(5.8046805746579E-17,6.86903940691701E-15,
-1.));
#130805=DIRECTION('ref_axis',(1.68321743785256E-34,-1.,-6.86903940691701E-15));
#130806=DIRECTION('',(-0.587785252292471,-0.809016994374949,-5.59128867158761E-15));
#130807=DIRECTION('center_axis',(-5.8046805746579E-17,-6.86903940691701E-15,
1.));
#130808=DIRECTION('ref_axis',(-2.17707695431367E-35,-1.,-6.86903940691701E-15));
#130809=DIRECTION('center_axis',(0.809016994374949,-0.587785252292471,-3.99055920848348E-15));
#130810=DIRECTION('ref_axis',(5.80468057465793E-17,6.86903940691702E-15,
-1.));
#130811=DIRECTION('center_axis',(0.809016994374951,-0.587785252292468,-1.46108553677859E-14));
#130812=DIRECTION('ref_axis',(0.514107226876147,0.707607892255898,0.484752338922551));
#130813=DIRECTION('',(-0.311481929006009,-0.428718095637372,-0.848044693619246));
#130814=DIRECTION('',(0.587785252292471,0.809016994374949,5.59128867158761E-15));
#130815=DIRECTION('',(-0.311481620848641,-0.428717671495144,0.848045021223099));
#130816=DIRECTION('center_axis',(0.809016994374939,-0.587785252292485,-3.92839125585453E-14));
#130817=DIRECTION('ref_axis',(0.514106124607336,0.707606375113047,-0.48475572254549));
#130818=DIRECTION('',(-0.587785252292471,-0.809016994374949,-5.73210557847752E-15));
#130819=DIRECTION('',(-0.293895572546214,-0.404512552559082,-0.866022509672739));
#130820=DIRECTION('center_axis',(-0.809016437837686,0.587786018297248,-1.63998888511843E-6));
#130821=DIRECTION('ref_axis',(0.509064546633241,0.7006672380552,0.499918702267869));
#130822=DIRECTION('',(-0.587785252292471,-0.809016994374949,-5.73210557847752E-15));
#130823=DIRECTION('center_axis',(-0.809017550961786,0.587784486213361,-1.64014389411998E-6));
#130824=DIRECTION('ref_axis',(0.509047470457493,0.700643735095407,-0.499969028333141));
#130825=DIRECTION('',(-0.293895664582667,-0.404512679236475,0.866022419268948));
#130826=DIRECTION('',(-0.587785252292471,-0.809016994374949,-5.73210557847752E-15));
#130827=DIRECTION('center_axis',(0.809016994374949,-0.587785252292471,-3.99055920848348E-15));
#130828=DIRECTION('ref_axis',(5.80468057465793E-17,6.86903940691702E-15,
-1.));
#130829=DIRECTION('center_axis',(-0.80901699437496,0.587785252292456,-5.37569329685675E-14));
#130830=DIRECTION('ref_axis',(0.514106124598334,0.707606375100633,-0.484755722573158));
#130831=DIRECTION('',(0.311481620848638,0.428717671495152,-0.848045021223095));
#130832=DIRECTION('',(-0.587785252292471,-0.809016994374949,-5.59128867158761E-15));
#130833=DIRECTION('',(0.311481929006021,0.428718095637366,0.848044693619245));
#130834=DIRECTION('center_axis',(-0.809016994374947,0.587785252292474,1.47486936277971E-14));
#130835=DIRECTION('ref_axis',(0.514107226887317,0.70760789227126,0.48475233888828));
#130836=DIRECTION('',(0.587785252292471,0.809016994374949,5.73210557847752E-15));
#130837=DIRECTION('',(0.293895664582692,0.40451267923646,-0.866022419268946));
#130838=DIRECTION('center_axis',(0.809016437708317,-0.587786018475307,-1.6403705029113E-6));
#130839=DIRECTION('ref_axis',(0.509064606990388,0.700667321129299,-0.499918524372936));
#130840=DIRECTION('',(0.587785252292471,0.809016994374949,5.73210557847752E-15));
#130841=DIRECTION('center_axis',(0.809017550837637,-0.587784486384239,-1.6397776906657E-6));
#130842=DIRECTION('ref_axis',(0.509047408032981,0.700643649175039,0.499969212297706));
#130843=DIRECTION('',(0.293895572546198,0.40451255255907,0.86602250967275));
#130844=DIRECTION('',(0.587785252292471,0.809016994374949,5.73210557847752E-15));
#130845=DIRECTION('center_axis',(-7.04084534449555E-17,-6.86101165903726E-15,
1.));
#130846=DIRECTION('ref_axis',(0.,-1.,-6.86101165903726E-15));
#130847=DIRECTION('',(0.499999999999998,0.86602540378444,5.97701461910997E-15));
#130848=DIRECTION('center_axis',(7.04084534449556E-17,6.86101165903726E-15,
-1.));
#130849=DIRECTION('ref_axis',(1.24809821036928E-34,-1.,-6.86101165903726E-15));
#130850=DIRECTION('',(-0.499999999999998,-0.86602540378444,-5.97701461910997E-15));
#130851=DIRECTION('center_axis',(-7.04084534449556E-17,-6.86101165903726E-15,
1.));
#130852=DIRECTION('ref_axis',(-7.43397775866882E-35,-1.,-6.86101165903726E-15));
#130853=DIRECTION('center_axis',(0.86602540378444,-0.499999999999998,-3.36953032019411E-15));
#130854=DIRECTION('ref_axis',(7.04084534449556E-17,6.86101165903726E-15,
-1.));
#130855=DIRECTION('center_axis',(0.866025403784421,-0.50000000000003,5.81677449547759E-14));
#130856=DIRECTION('ref_axis',(0.437325728121601,0.757470380563662,0.484752338923344));
#130857=DIRECTION('',(-0.264962354696014,-0.458928260426592,-0.848044693619249));
#130858=DIRECTION('',(0.499999999999998,0.86602540378444,5.97701461910997E-15));
#130859=DIRECTION('',(-0.264962092561698,-0.458927806396633,0.848045021223108));
#130860=DIRECTION('center_axis',(0.86602540378445,-0.49999999999998,3.34947043920223E-14));
#130861=DIRECTION('ref_axis',(0.437324790476197,0.757468756514194,-0.484755722544655));
#130862=DIRECTION('',(-0.499999999999998,-0.86602540378444,-6.11783152599987E-15));
#130863=DIRECTION('',(-0.250002506357479,-0.433017043030743,-0.866022509672751));
#130864=DIRECTION('center_axis',(-0.866024930365256,0.500000819982492,-1.63998893916804E-6));
#130865=DIRECTION('ref_axis',(0.433036168126024,0.750040644375844,0.499918702269678));
#130866=DIRECTION('',(-0.499999999999998,-0.86602540378444,-6.11783152599987E-15));
#130867=DIRECTION('center_axis',(-0.866025877245197,0.499999179938324,-1.64014403630087E-6));
#130868=DIRECTION('ref_axis',(0.433021642223467,0.750015485220938,-0.499969028335648));
#130869=DIRECTION('',(-0.250002584648417,-0.433017178634595,0.866022419268951));
#130870=DIRECTION('',(-0.499999999999998,-0.86602540378444,-6.11783152599987E-15));
#130871=DIRECTION('center_axis',(0.86602540378444,-0.499999999999998,-3.36953032019411E-15));
#130872=DIRECTION('ref_axis',(7.04084534449556E-17,6.86101165903726E-15,
-1.));
#130873=DIRECTION('center_axis',(-0.86602540378442,0.500000000000033,5.65136987618391E-14));
#130874=DIRECTION('ref_axis',(0.43732479046754,0.757468756499181,-0.484755722575925));
#130875=DIRECTION('',(0.264962092561698,0.458927806396633,-0.848045021223108));
#130876=DIRECTION('',(-0.499999999999998,-0.86602540378444,-5.97701461910997E-15));
#130877=DIRECTION('',(0.264962354696018,0.458928260426587,0.84804469361925));
#130878=DIRECTION('center_axis',(-0.866025403784437,0.500000000000003,2.48108864766678E-15));
#130879=DIRECTION('ref_axis',(0.437325728131431,0.757470380580684,0.484752338887877));
#130880=DIRECTION('',(0.499999999999998,0.86602540378444,6.11783152599988E-15));
#130881=DIRECTION('',(0.250002584648414,0.43301717863459,-0.866022419268954));
#130882=DIRECTION('center_axis',(0.866024930255218,-0.500000820173081,-1.64037040324638E-6));
#130883=DIRECTION('ref_axis',(0.433036219468666,0.750040733303334,-0.499918524375804));
#130884=DIRECTION('',(0.499999999999998,0.86602540378444,6.11783152599987E-15));
#130885=DIRECTION('center_axis',(0.866025877139533,-0.499999180121342,-1.63977762112504E-6));
#130886=DIRECTION('ref_axis',(0.433021589122546,0.750015393246993,0.499969212298461));
#130887=DIRECTION('',(0.250002506357474,0.433017043030739,0.866022509672755));
#130888=DIRECTION('',(0.499999999999998,0.86602540378444,6.11783152599987E-15));
#130889=DIRECTION('center_axis',(-8.35415108931911E-17,-6.85432003203771E-15,
1.));
#130890=DIRECTION('ref_axis',(0.,-1.,-6.85432003203771E-15));
#130891=DIRECTION('',(0.406736643075798,0.913545457642602,6.29571232419492E-15));
#130892=DIRECTION('center_axis',(8.35415108931911E-17,6.85432003203771E-15,
-1.));
#130893=DIRECTION('ref_axis',(1.65551687784934E-34,-1.,-6.85432003203771E-15));
#130894=DIRECTION('',(-0.406736643075798,-0.913545457642602,-6.29571232419492E-15));
#130895=DIRECTION('center_axis',(-8.35415108931911E-17,-6.85432003203771E-15,
1.));
#130896=DIRECTION('ref_axis',(-3.34580098672039E-35,-1.,-6.85432003203771E-15));
#130897=DIRECTION('center_axis',(0.913545457642602,-0.406736643075798,-2.71158415259714E-15));
#130898=DIRECTION('ref_axis',(8.35415108931909E-17,6.85432003203771E-15,
-1.));
#130899=DIRECTION('center_axis',(0.913545457642599,-0.406736643075804,8.27029549119894E-16));
#130900=DIRECTION('ref_axis',(0.355752797174059,0.799033864872216,0.484752338921848));
#130901=DIRECTION('',(-0.215539797381028,-0.48411031115768,-0.848044693619246));
#130902=DIRECTION('',(0.406736643075798,0.913545457642602,6.29571232419492E-15));
#130903=DIRECTION('',(-0.215539584141774,-0.484109832214441,0.848045021223105));
#130904=DIRECTION('center_axis',(0.913545457642602,-0.406736643075797,6.89191448395568E-16));
#130905=DIRECTION('ref_axis',(0.355752034424597,0.79903215170889,-0.484755722543036));
#130906=DIRECTION('',(-0.406736643075798,-0.913545457642602,-6.43652923108483E-15));
#130907=DIRECTION('',(-0.203370360392777,-0.45677730816434,-0.866022509672729));
#130908=DIRECTION('center_axis',(-0.913545072528373,0.406737508052111,-1.63998884914257E-6));
#130909=DIRECTION('ref_axis',(0.352263354743096,0.791196448441969,0.499918702268634));
#130910=DIRECTION('',(-0.406736643075798,-0.913545457642602,-6.43652923108483E-15));
#130911=DIRECTION('center_axis',(-0.91354584278991,0.406735778016372,-1.64014401684982E-6));
#130912=DIRECTION('ref_axis',(0.352251538263059,0.791169908742093,-0.499969028333092));
#130913=DIRECTION('',(-0.203370424080347,-0.456777451208944,0.866022419268947));
#130914=DIRECTION('',(-0.406736643075798,-0.913545457642602,-6.43652923108483E-15));
#130915=DIRECTION('center_axis',(0.913545457642602,-0.406736643075798,-2.71158415259714E-15));
#130916=DIRECTION('ref_axis',(8.35415108931909E-17,6.85432003203771E-15,
-1.));
#130917=DIRECTION('center_axis',(-0.913545457642604,0.406736643075794,-2.48108921393404E-15));
#130918=DIRECTION('ref_axis',(0.355752034417932,0.799032151693926,-0.484755722572594));
#130919=DIRECTION('',(0.215539584141771,0.484109832214462,-0.848045021223094));
#130920=DIRECTION('',(-0.406736643075798,-0.913545457642602,-6.29571232419492E-15));
#130921=DIRECTION('',(0.215539797381042,0.484110311157681,0.848044693619241));
#130922=DIRECTION('center_axis',(-0.913545457642596,0.40673664307581,-1.51622084024078E-14));
#130923=DIRECTION('ref_axis',(0.355752797181947,0.799033864889936,0.48475233888685));
#130924=DIRECTION('',(0.406736643075798,0.913545457642602,6.43652923108483E-15));
#130925=DIRECTION('',(0.203370424080339,0.456777451208961,-0.866022419268941));
#130926=DIRECTION('center_axis',(0.913545072438839,-0.406737508253204,-1.64037044800086E-6));
#130927=DIRECTION('ref_axis',(0.352263396508499,0.79119654224795,-0.499918524376906));
#130928=DIRECTION('',(0.406736643075798,0.913545457642602,6.43652923108483E-15));
#130929=DIRECTION('center_axis',(0.913545842703945,-0.406735778209453,-1.63977757413235E-6));
#130930=DIRECTION('ref_axis',(0.352251495067333,0.791169811722332,0.499969212294195));
#130931=DIRECTION('',(0.203370360392769,0.456777308164283,0.866022509672761));
#130932=DIRECTION('',(0.406736643075798,0.913545457642602,6.43652923108483E-15));
#130933=DIRECTION('center_axis',(-9.73020895656139E-17,-6.84903784078409E-15,
1.));
#130934=DIRECTION('ref_axis',(0.,-1.,-6.84903784078409E-15));
#130935=DIRECTION('',(0.309016994374945,0.951056516295154,6.54389006809377E-15));
#130936=DIRECTION('center_axis',(9.73020895656139E-17,6.84903784078409E-15,
-1.));
#130937=DIRECTION('ref_axis',(-3.21147635721861E-34,-1.,-6.84903784078409E-15));
#130938=DIRECTION('',(-0.309016994374945,-0.951056516295154,-6.54389006809377E-15));
#130939=DIRECTION('center_axis',(-9.73020895656139E-17,-6.84903784078409E-15,
1.));
#130940=DIRECTION('ref_axis',(1.61937966168246E-34,-1.,-6.84903784078409E-15));
#130941=DIRECTION('center_axis',(0.951056516295154,-0.309016994374945,-2.02392930158885E-15));
#130942=DIRECTION('ref_axis',(9.73020895656142E-17,6.84903784078409E-15,
-1.));
#130943=DIRECTION('center_axis',(0.951056516295153,-0.30901699437495,1.32324727859198E-14));
#130944=DIRECTION('ref_axis',(0.270282164134238,0.831842966948057,0.484752338921605));
#130945=DIRECTION('',(-0.163755740941347,-0.503988348013117,-0.848044693619246));
#130946=DIRECTION('',(0.309016994374945,0.951056516295154,6.54389006809377E-15));
#130947=DIRECTION('',(-0.163755578933429,-0.50398784940401,0.848045021223106));
#130948=DIRECTION('center_axis',(0.951056516295158,-0.309016994374936,1.46108587059839E-14));
#130949=DIRECTION('ref_axis',(0.270281584637381,0.831841183440119,-0.484755722543684));
#130950=DIRECTION('',(-0.309016994374945,-0.951056516295154,-6.68470697498368E-15));
#130951=DIRECTION('',(-0.154510046201584,-0.47553302552284,-0.866022509672744));
#130952=DIRECTION('center_axis',(-0.951056223705258,0.309017894868251,-1.63998889432737E-6));
#130953=DIRECTION('ref_axis',(0.26763107032928,0.823683738649504,0.499918702269459));
#130954=DIRECTION('',(-0.309016994374945,-0.951056516295154,-6.68470697498368E-15));
#130955=DIRECTION('center_axis',(-0.951056808909242,0.309016093795583,-1.6401439545386E-6));
#130956=DIRECTION('ref_axis',(0.267622092735265,0.823656109178587,-0.499969028333544));
#130957=DIRECTION('',(-0.154510094588056,-0.475533174441008,0.866022419268952));
#130958=DIRECTION('',(-0.309016994374945,-0.951056516295154,-6.68470697498368E-15));
#130959=DIRECTION('center_axis',(0.951056516295154,-0.309016994374945,-2.02392930158885E-15));
#130960=DIRECTION('ref_axis',(9.73020895656142E-17,6.84903784078409E-15,
-1.));
#130961=DIRECTION('center_axis',(-0.951056516295147,0.309016994374967,3.33568660984485E-14));
#130962=DIRECTION('ref_axis',(0.270281584632204,0.83184118342417,-0.484755722573938));
#130963=DIRECTION('',(0.16375557893343,0.503987849404014,-0.848045021223103));
#130964=DIRECTION('',(-0.309016994374945,-0.951056516295154,-6.54389006809377E-15));
#130965=DIRECTION('',(0.16375574094134,0.503988348013127,0.848044693619241));
#130966=DIRECTION('center_axis',(-0.951056516295154,0.309016994374946,5.7892068445558E-15));
#130967=DIRECTION('ref_axis',(0.270282164140123,0.831842966966152,0.484752338887273));
#130968=DIRECTION('',(0.309016994374945,0.951056516295154,6.68470697498368E-15));
#130969=DIRECTION('',(0.154510094588052,0.47553317444103,-0.86602241926894));
#130970=DIRECTION('center_axis',(0.951056223637263,-0.309017895077515,-1.64037034454954E-6));
#130971=DIRECTION('ref_axis',(0.267631102061259,0.823683836309653,-0.499918524373411));
#130972=DIRECTION('',(0.309016994374945,0.951056516295154,6.68470697498368E-15));
#130973=DIRECTION('center_axis',(0.951056808843944,-0.30901609399655,-1.63977759461637E-6));
#130974=DIRECTION('ref_axis',(0.267622059916621,0.823656008172419,0.499969212299579));
#130975=DIRECTION('',(0.154510046201588,0.475533025522823,0.866022509672753));
#130976=DIRECTION('',(0.309016994374945,0.951056516295154,6.68470697498368E-15));
#130977=DIRECTION('center_axis',(-1.11539425682703E-16,-6.84522295806915E-15,
1.));
#130978=DIRECTION('ref_axis',(0.,-1.,-6.84522295806915E-15));
#130979=DIRECTION('',(0.207911690817756,0.978147600733806,6.71882876350984E-15));
#130980=DIRECTION('center_axis',(1.11539425682703E-16,6.84522295806915E-15,
-1.));
#130981=DIRECTION('ref_axis',(-2.39543546274231E-35,-1.,-6.84522295806915E-15));
#130982=DIRECTION('',(-0.207911690817756,-0.978147600733806,-6.71882876350984E-15));
#130983=DIRECTION('center_axis',(-1.11539425682703E-16,-6.84522295806915E-15,
1.));
#130984=DIRECTION('ref_axis',(-2.39876940632517E-34,-1.,-6.84522295806915E-15));
#130985=DIRECTION('center_axis',(0.978147600733806,-0.207911690817756,-1.31409985761792E-15));
#130986=DIRECTION('ref_axis',(1.11539425682703E-16,6.84522295806915E-15,
-1.));
#130987=DIRECTION('center_axis',(0.978147600733806,-0.207911690817757,1.03378693639992E-14));
#130988=DIRECTION('ref_axis',(0.181850263143883,0.855538223403326,0.484752338922033));
#130989=DIRECTION('',(-0.110177542335811,-0.518344583061382,-0.848044693619247));
#130990=DIRECTION('',(0.207911690817756,0.978147600733806,6.71882876350984E-15));
#130991=DIRECTION('',(-0.110177433334227,-0.518344070249277,0.848045021223104));
#130992=DIRECTION('center_axis',(0.978147600733807,-0.207911690817751,-2.06757434518653E-16));
#130993=DIRECTION('ref_axis',(0.181849873248985,0.85553638909205,-0.484755722543494));
#130994=DIRECTION('',(-0.207911690817756,-0.978147600733806,-6.85964567039975E-15));
#130995=DIRECTION('',(-0.103956887610937,-0.48907870354206,-0.866022509672737));
#130996=DIRECTION('center_axis',(-0.978147403873936,0.207912616962008,-1.6399888600733E-6));
#130997=DIRECTION('ref_axis',(0.180066563903243,0.847146577447699,0.49991870227341));
#130998=DIRECTION('',(-0.207911690817756,-0.978147600733806,-6.85964567039975E-15));
#130999=DIRECTION('center_axis',(-0.978147797608753,0.207910764585331,-1.64014399602197E-6));
#131000=DIRECTION('ref_axis',(0.180060523556148,0.847118160922542,-0.499969028332651));
#131001=DIRECTION('',(-0.103956920166139,-0.489078856702179,0.866022419268959));
#131002=DIRECTION('',(-0.207911690817756,-0.978147600733806,-6.85964567039975E-15));
#131003=DIRECTION('center_axis',(0.978147600733806,-0.207911690817756,-1.31409985761792E-15));
#131004=DIRECTION('ref_axis',(1.11539425682703E-16,6.84522295806915E-15,
-1.));
#131005=DIRECTION('center_axis',(-0.978147600733803,0.20791169081777,9.51084198674763E-15));
#131006=DIRECTION('ref_axis',(0.181849873245726,0.855536389076659,-0.484755722571879));
#131007=DIRECTION('',(0.110177433334223,0.518344070249286,-0.848045021223099));
#131008=DIRECTION('',(-0.207911690817756,-0.978147600733806,-6.71882876350983E-15));
#131009=DIRECTION('',(0.110177542335811,0.518344583061368,0.848044693619255));
#131010=DIRECTION('center_axis',(-0.978147600733808,0.20791169081775,3.79055210060189E-15));
#131011=DIRECTION('ref_axis',(0.18185026314782,0.855538223421847,0.484752338887868));
#131012=DIRECTION('',(0.207911690817756,0.978147600733806,6.85964567039975E-15));
#131013=DIRECTION('',(0.103956920166119,0.489078856702167,-0.866022419268968));
#131014=DIRECTION('center_axis',(0.978147403828172,-0.207912617177303,-1.64037042906602E-6));
#131015=DIRECTION('ref_axis',(0.180066585253188,0.847146677890037,-0.499918524376853));
#131016=DIRECTION('',(0.207911690817756,0.978147600733806,6.85964567039975E-15));
#131017=DIRECTION('center_axis',(0.978147797564806,-0.207910764792088,-1.63977754134118E-6));
#131018=DIRECTION('ref_axis',(0.18006050147535,0.847118057039365,0.499969212298413));
#131019=DIRECTION('',(0.103956887610919,0.489078703542023,0.86602250967276));
#131020=DIRECTION('',(0.207911690817756,0.978147600733806,6.85964567039975E-15));
#131021=DIRECTION('center_axis',(-1.26097532010604E-16,-6.84291718054622E-15,
1.));
#131022=DIRECTION('ref_axis',(0.,-1.,-6.84291718054622E-15));
#131023=DIRECTION('',(0.10452846326765,0.994521895368274,6.81861174548786E-15));
#131024=DIRECTION('center_axis',(1.26097532010604E-16,6.84291718054622E-15,
-1.));
#131025=DIRECTION('ref_axis',(-3.1783372781003E-34,-1.,-6.84291718054621E-15));
#131026=DIRECTION('',(-0.10452846326765,-0.994521895368274,-6.81861174548786E-15));
#131027=DIRECTION('center_axis',(-1.26097532010604E-16,-6.84291718054622E-15,
1.));
#131028=DIRECTION('ref_axis',(3.64495957293817E-34,-1.,-6.84291718054622E-15));
#131029=DIRECTION('center_axis',(0.994521895368274,-0.10452846326765,-5.89872860613851E-16));
#131030=DIRECTION('ref_axis',(1.26097532010604E-16,6.84291718054622E-15,
-1.));
#131031=DIRECTION('center_axis',(0.994521895368275,-0.10452846326764,-2.22608786971444E-14));
#131032=DIRECTION('ref_axis',(0.0914259726159116,0.869860024049565,0.484752338923418));
#131033=DIRECTION('',(-0.0553922155203051,-0.527021726387053,-0.848044693619247));
#131034=DIRECTION('',(0.10452846326765,0.994521895368274,6.81861174548786E-15));
#131035=DIRECTION('',(-0.0553921607193105,-0.527021204990399,0.848045021223115));
#131036=DIRECTION('center_axis',(0.994521895368273,-0.104528463267657,-1.44041012714673E-14));
#131037=DIRECTION('ref_axis',(0.0914257765946934,0.86985815903228,-0.48475572254387));
#131038=DIRECTION('',(-0.10452846326765,-0.994521895368274,-6.95942865237777E-15));
#131039=DIRECTION('',(-0.0522647556052144,-0.497265932938934,-0.866022509672756));
#131040=DIRECTION('center_axis',(-0.994521796395255,0.104529404915866,-1.63998886226799E-6));
#131041=DIRECTION('ref_axis',(0.090529210522719,0.861327901071179,0.499918702269129));
#131042=DIRECTION('',(-0.10452846326765,-0.994521895368274,-6.95942865237777E-15));
#131043=DIRECTION('center_axis',(-0.994521994347068,0.104527521530168,-1.64014403750577E-6));
#131044=DIRECTION('ref_axis',(0.0905261736004185,0.861299008821256,-0.499969028337546));
#131045=DIRECTION('',(-0.0522647719724818,-0.49726608866303,0.866022419268945));
#131046=DIRECTION('',(-0.10452846326765,-0.994521895368274,-6.95942865237777E-15));
#131047=DIRECTION('center_axis',(0.994521895368274,-0.10452846326765,-5.89872860613851E-16));
#131048=DIRECTION('ref_axis',(1.26097532010604E-16,6.84291718054622E-15,
-1.));
#131049=DIRECTION('center_axis',(-0.994521895368273,0.104528463267658,6.61623790382405E-15));
#131050=DIRECTION('ref_axis',(0.0914257765928784,0.869858159014973,-0.484755722575269));
#131051=DIRECTION('',(0.0553921607193085,0.527021204990422,-0.848045021223101));
#131052=DIRECTION('',(-0.10452846326765,-0.994521895368274,-6.81861174548786E-15));
#131053=DIRECTION('',(0.0553922155203075,0.527021726387058,0.848044693619244));
#131054=DIRECTION('center_axis',(-0.994521895368274,0.104528463267647,9.13178460599565E-15));
#131055=DIRECTION('ref_axis',(0.0914259726180026,0.86986002406946,0.484752338887324));
#131056=DIRECTION('',(0.10452846326765,0.994521895368274,6.95942865237777E-15));
#131057=DIRECTION('',(0.0522647719724739,0.497266088663004,-0.86602241926896));
#131058=DIRECTION('center_axis',(0.994521796372252,-0.104529405134716,-1.6403703829347E-6));
#131059=DIRECTION('ref_axis',(0.0905292212565932,0.861328003194837,-0.499918524372793));
#131060=DIRECTION('',(0.10452846326765,0.994521895368274,6.95942865237777E-15));
#131061=DIRECTION('center_axis',(0.994521994324978,-0.104527521740355,-1.63977761557319E-6));
#131062=DIRECTION('ref_axis',(0.0905261624997722,0.861298903203399,0.499969212295804));
#131063=DIRECTION('',(0.0522647556052142,0.497265932938926,0.866022509672761));
#131064=DIRECTION('',(0.10452846326765,0.994521895368274,6.95942865237777E-15));
#131065=DIRECTION('center_axis',(-1.40816906889911E-16,-6.84214577079636E-15,
1.));
#131066=DIRECTION('ref_axis',(-1.,9.8331920519947E-31,-1.40816906889911E-16));
#131067=DIRECTION('',(-3.49148133884313E-15,1.,6.84214577079636E-15));
#131068=DIRECTION('center_axis',(1.40816906889911E-16,6.84214577079636E-15,
-1.));
#131069=DIRECTION('ref_axis',(-1.,1.19595411430356E-30,-1.40816906889911E-16));
#131070=DIRECTION('',(3.49148133884313E-15,-1.,-6.84214577079636E-15));
#131071=DIRECTION('center_axis',(-1.40816906889911E-16,-6.84214577079636E-15,
1.));
#131072=DIRECTION('ref_axis',(-1.,8.43631878914075E-31,-1.40816906889911E-16));
#131073=DIRECTION('center_axis',(1.,3.49148133884313E-15,1.40816906889935E-16));
#131074=DIRECTION('ref_axis',(1.40816906889911E-16,6.84214577079636E-15,
-1.));
#131075=DIRECTION('center_axis',(1.,3.44043747061122E-15,3.3107378020012E-16));
#131076=DIRECTION('ref_axis',(-3.16967243309519E-15,0.87465145624433,0.484752338921301));
#131077=DIRECTION('',(1.96084725663078E-15,-0.52992470939204,-0.848044693619247));
#131078=DIRECTION('',(-3.49148133884313E-15,1.,6.84214577079636E-15));
#131079=DIRECTION('',(1.75444295999835E-15,-0.529924185123399,0.848045021223108));
#131080=DIRECTION('center_axis',(1.,3.58452992681197E-15,2.19445148712543E-16));
#131081=DIRECTION('ref_axis',(-3.02883030677592E-15,0.874649580952794,-0.484755722543945));
#131082=DIRECTION('',(3.49148133884313E-15,-1.,-6.98296267768627E-15));
#131083=DIRECTION('',(1.92690513386524E-15,-0.500005012715014,-0.866022509672733));
#131084=DIRECTION('center_axis',(-0.999999999998207,9.46835254807534E-7,
-1.639988859514E-6));
#131085=DIRECTION('ref_axis',(1.66718524320421E-10,0.866072335964842,0.49991870226708));
#131086=DIRECTION('',(3.49148133884313E-15,-1.,-6.98296267768627E-15));
#131087=DIRECTION('center_axis',(-0.999999999998207,-9.46924665087402E-7,
-1.64014406431857E-6));
#131088=DIRECTION('ref_axis',(-5.65130087085307E-11,0.866043284546834,-0.499969028332087));
#131089=DIRECTION('',(1.51399673284832E-15,-0.50000516929684,0.866022419268946));
#131090=DIRECTION('',(3.49148133884313E-15,-1.,-6.98296267768627E-15));
#131091=DIRECTION('center_axis',(1.,3.49148133884313E-15,1.40816906889935E-16));
#131092=DIRECTION('ref_axis',(1.40816906889911E-16,6.84214577079636E-15,
-1.));
#131093=DIRECTION('center_axis',(-1.,-3.31723128487435E-15,2.6278067191977E-16));
#131094=DIRECTION('ref_axis',(-3.02879938767599E-15,0.874649580935239,-0.48475572257562));
#131095=DIRECTION('',(-1.702841696469E-15,0.529924185123403,-0.848045021223106));
#131096=DIRECTION('',(3.49148133884313E-15,-1.,-6.84214577079636E-15));
#131097=DIRECTION('',(-1.90924601303524E-15,0.52992470939203,0.848044693619253));
#131098=DIRECTION('center_axis',(-1.,-3.24518402866521E-15,-5.38039174125174E-16));
#131099=DIRECTION('ref_axis',(-3.09922068458486E-15,0.874651456263469,0.48475233888677));
#131100=DIRECTION('',(-3.49148133884313E-15,1.,6.98296267768627E-15));
#131101=DIRECTION('',(-1.6516327994709E-15,0.50000516929684,-0.866022419268946));
#131102=DIRECTION('center_axis',(0.999999999998206,-9.47055338026444E-7,
-1.64037041142286E-6));
#131103=DIRECTION('ref_axis',(1.6697062825775E-10,0.866072438647394,-0.499918524377079));
#131104=DIRECTION('',(-3.49148133884313E-15,1.,6.98296267768627E-15));
#131105=DIRECTION('center_axis',(0.999999999998207,9.46713294510181E-7,
-1.63977760303538E-6));
#131106=DIRECTION('ref_axis',(-5.62740263084214E-11,0.866043178343555,0.499969212296711));
#131107=DIRECTION('',(-1.92690513386528E-15,0.500005012714987,0.866022509672748));
#131108=DIRECTION('',(-3.49148133884313E-15,1.,6.98296267768627E-15));
#131109=DIRECTION('center_axis',(-1.55536281769218E-16,-6.84291718054622E-15,
1.));
#131110=DIRECTION('ref_axis',(-1.,1.08610405062054E-30,-1.55536281769218E-16));
#131111=DIRECTION('',(-0.104528463267657,0.994521895368273,6.78917299572924E-15));
#131112=DIRECTION('center_axis',(1.55536281769218E-16,6.84291718054622E-15,
-1.));
#131113=DIRECTION('ref_axis',(-1.,1.15501815782576E-30,-1.55536281769218E-16));
#131114=DIRECTION('',(0.104528463267657,-0.994521895368273,-6.78917299572924E-15));
#131115=DIRECTION('center_axis',(-1.55536281769218E-16,-6.84291718054622E-15,
1.));
#131116=DIRECTION('ref_axis',(-1.,1.26143365054205E-30,-1.55536281769218E-16));
#131117=DIRECTION('center_axis',(0.994521895368273,0.104528463267657,8.69963854894001E-16));
#131118=DIRECTION('ref_axis',(1.55536281769218E-16,6.84291718054622E-15,
-1.));
#131119=DIRECTION('center_axis',(0.994521895368273,0.10452846326766,-6.61623639296017E-15));
#131120=DIRECTION('ref_axis',(0.0914259726160256,-0.869860024050614,-0.484752338921515));
#131121=DIRECTION('',(0.0553922155203091,-0.527021726387057,-0.848044693619244));
#131122=DIRECTION('',(-0.104528463267657,0.994521895368273,6.78917299572924E-15));
#131123=DIRECTION('',(0.0553921607193154,-0.527021204990399,0.848045021223115));
#131124=DIRECTION('center_axis',(0.994521895368271,0.104528463267677,4.04899975932421E-14));
#131125=DIRECTION('ref_axis',(0.0914257765946187,-0.869858159031526,0.484755722545237));
#131126=DIRECTION('',(0.104528463267657,-0.994521895368273,-6.92998990261915E-15));
#131127=DIRECTION('',(0.0522647556052223,-0.497265932938961,-0.86602250967274));
#131128=DIRECTION('center_axis',(-0.994521994337723,-0.104527521619084,
-1.63998884823934E-6));
#131129=DIRECTION('ref_axis',(0.0905292101911854,-0.861327901106789,-0.499918702267812));
#131130=DIRECTION('',(0.104528463267657,-0.994521895368273,-6.92998990261915E-15));
#131131=DIRECTION('center_axis',(-0.994521796385912,-0.104529405004756,
-1.64014403298725E-6));
#131132=DIRECTION('ref_axis',(0.0905261737132939,-0.861299008813934,0.499969028329721));
#131133=DIRECTION('',(0.0522647719724805,-0.497266088663018,0.866022419268952));
#131134=DIRECTION('',(0.104528463267657,-0.994521895368273,-6.92998990261915E-15));
#131135=DIRECTION('center_axis',(0.994521895368273,0.104528463267657,8.69963854894001E-16));
#131136=DIRECTION('ref_axis',(1.55536281769218E-16,6.84291718054622E-15,
-1.));
#131137=DIRECTION('center_axis',(-0.994521895368273,-0.104528463267655,
3.58379553123804E-15));
#131138=DIRECTION('ref_axis',(0.0914257765929169,-0.869858159015314,0.484755722574649));
#131139=DIRECTION('',(-0.0553921607193138,0.527021204990413,-0.848045021223107));
#131140=DIRECTION('',(0.104528463267657,-0.994521895368273,-6.78917299572924E-15));
#131141=DIRECTION('',(-0.0553922155203088,0.527021726387043,0.848044693619253));
#131142=DIRECTION('center_axis',(-0.994521895368272,-0.104528463267666,
1.06480054462366E-14));
#131143=DIRECTION('ref_axis',(0.091425972617933,-0.869860024068733,-0.484752338888641));
#131144=DIRECTION('',(-0.104528463267657,0.994521895368273,6.92998990261915E-15));
#131145=DIRECTION('',(-0.0522647719724874,0.497266088663041,-0.866022419268938));
#131146=DIRECTION('center_axis',(0.994521994360729,0.104527521400187,-1.64037042071753E-6));
#131147=DIRECTION('ref_axis',(0.0905292209241164,-0.861328003226279,0.499918524378826));
#131148=DIRECTION('',(-0.104528463267657,0.994521895368273,6.92998990261915E-15));
#131149=DIRECTION('center_axis',(0.994521796408008,0.10452940479454,-1.63977756432044E-6));
#131150=DIRECTION('ref_axis',(0.0905261626117495,-0.861298903192075,-0.499969212295037));
#131151=DIRECTION('',(-0.0522647556052286,0.497265932938937,0.866022509672754));
#131152=DIRECTION('',(-0.104528463267657,0.994521895368273,6.92998990261915E-15));
#131153=DIRECTION('center_axis',(-1.70094388097119E-16,-6.84522295806915E-15,
1.));
#131154=DIRECTION('ref_axis',(-1.,1.18776276376607E-30,-1.70094388097119E-16));
#131155=DIRECTION('',(-0.207911690817763,0.978147600733805,6.66027380109541E-15));
#131156=DIRECTION('center_axis',(1.70094388097119E-16,6.84522295806915E-15,
-1.));
#131157=DIRECTION('ref_axis',(-1.,1.16019143467152E-30,-1.70094388097119E-16));
#131158=DIRECTION('',(0.207911690817763,-0.978147600733805,-6.66027380109541E-15));
#131159=DIRECTION('center_axis',(-1.70094388097119E-16,-6.84522295806915E-15,
1.));
#131160=DIRECTION('ref_axis',(-1.,1.26050675734334E-30,-1.70094388097119E-16));
#131161=DIRECTION('center_axis',(0.978147600733805,0.207911690817763,1.58957929685221E-15));
#131162=DIRECTION('ref_axis',(1.70094388097119E-16,6.84522295806915E-15,
-1.));
#131163=DIRECTION('center_axis',(0.978147600733804,0.207911690817767,-2.12270917607467E-14));
#131164=DIRECTION('ref_axis',(0.181850263143777,-0.855538223402809,-0.484752338922984));
#131165=DIRECTION('',(0.110177542335814,-0.518344583061392,-0.848044693619241));
#131166=DIRECTION('',(-0.207911690817763,0.978147600733805,6.66027380109541E-15));
#131167=DIRECTION('',(0.110177433334229,-0.518344070249262,0.848045021223113));
#131168=DIRECTION('center_axis',(0.978147600733799,0.207911690817789,5.18271969193474E-14));
#131169=DIRECTION('ref_axis',(0.181849873249002,-0.855536389092088,0.484755722543421));
#131170=DIRECTION('',(0.207911690817763,-0.978147600733805,-6.80109070798532E-15));
#131171=DIRECTION('',(0.103956887610948,-0.489078703542072,-0.866022509672728));
#131172=DIRECTION('center_axis',(-0.97814779759017,-0.207910764672759,-1.63998884285995E-6));
#131173=DIRECTION('ref_axis',(0.180066563577228,-0.847146577517634,-0.499918702272328));
#131174=DIRECTION('',(0.207911690817763,-0.978147600733805,-6.80109070798532E-15));
#131175=DIRECTION('center_axis',(-0.97814740385534,-0.207912617049492,-1.6401440806252E-6));
#131176=DIRECTION('ref_axis',(0.180060523666301,-0.847118160897096,0.499969028336096));
#131177=DIRECTION('',(0.103956920166122,-0.48907885670218,0.866022419268961));
#131178=DIRECTION('',(0.207911690817763,-0.978147600733805,-6.80109070798532E-15));
#131179=DIRECTION('center_axis',(0.978147600733805,0.207911690817763,1.58957929685221E-15));
#131180=DIRECTION('ref_axis',(1.70094388097119E-16,6.84522295806915E-15,
-1.));
#131181=DIRECTION('center_axis',(-0.978147600733801,-0.207911690817782,
-2.26054795047341E-14));
#131182=DIRECTION('ref_axis',(0.181849873245555,-0.855536389075835,0.484755722573397));
#131183=DIRECTION('',(-0.110177433334229,0.518344070249272,-0.848045021223107));
#131184=DIRECTION('',(0.207911690817763,-0.978147600733805,-6.66027380109541E-15));
#131185=DIRECTION('',(-0.110177542335816,0.518344583061377,0.84804469361925));
#131186=DIRECTION('center_axis',(-0.978147600733805,-0.207911690817762,
9.0284059123426E-15));
#131187=DIRECTION('ref_axis',(0.181850263147824,-0.855538223421843,-0.484752338887874));
#131188=DIRECTION('',(-0.207911690817763,0.978147600733805,6.80109070798532E-15));
#131189=DIRECTION('',(-0.10395692016612,0.489078856702206,-0.866022419268946));
#131190=DIRECTION('center_axis',(0.978147797635921,0.20791076445751,-1.64037035642678E-6));
#131191=DIRECTION('ref_axis',(0.180066584926945,-0.847146677961353,0.499918524373514));
#131192=DIRECTION('',(-0.207911690817763,0.978147600733805,6.80109070798532E-15));
#131193=DIRECTION('center_axis',(0.978147403899296,0.207912616842697,-1.63977756113648E-6));
#131194=DIRECTION('ref_axis',(0.180060501585272,-0.847118057015218,-0.49996921229974));
#131195=DIRECTION('',(-0.103956887610925,0.489078703542011,0.866022509672765));
#131196=DIRECTION('',(-0.207911690817763,0.978147600733805,6.80109070798532E-15));
#131197=DIRECTION('center_axis',(-1.84331724214208E-16,-6.84903784078409E-15,
1.));
#131198=DIRECTION('ref_axis',(-1.,1.28718155050137E-30,-1.84331724214208E-16));
#131199=DIRECTION('',(-0.309016994374951,0.951056516295152,6.45686043344516E-15));
#131200=DIRECTION('center_axis',(1.84331724214208E-16,6.84903784078409E-15,
-1.));
#131201=DIRECTION('ref_axis',(-1.,1.16316872187192E-30,-1.84331724214208E-16));
#131202=DIRECTION('',(0.309016994374951,-0.951056516295152,-6.45686043344516E-15));
#131203=DIRECTION('center_axis',(-1.84331724214208E-16,-6.84903784078409E-15,
1.));
#131204=DIRECTION('ref_axis',(-1.,1.25738374682677E-30,-1.84331724214208E-16));
#131205=DIRECTION('center_axis',(0.951056516295152,0.309016994374951,2.29177897539325E-15));
#131206=DIRECTION('ref_axis',(1.84331724214208E-16,6.84903784078409E-15,
-1.));
#131207=DIRECTION('center_axis',(0.951056516295154,0.309016994374946,2.1778444793492E-14));
#131208=DIRECTION('ref_axis',(0.270282164134052,-0.831842966947439,-0.484752338922769));
#131209=DIRECTION('',(0.163755740941359,-0.503988348013111,-0.848044693619247));
#131210=DIRECTION('',(-0.309016994374951,0.951056516295152,6.45686043344516E-15));
#131211=DIRECTION('',(0.163755578933428,-0.50398784940402,0.848045021223101));
#131212=DIRECTION('center_axis',(0.951056516295148,0.309016994374966,3.11514534674777E-14));
#131213=DIRECTION('ref_axis',(0.270281584637533,-0.831841183440571,0.484755722542823));
#131214=DIRECTION('',(0.309016994374951,-0.951056516295152,-6.59767734033507E-15));
#131215=DIRECTION('',(0.154510046201604,-0.475533025522845,-0.866022509672738));
#131216=DIRECTION('center_axis',(-0.951056808881636,-0.309016093880544,
-1.63998884845428E-6));
#131217=DIRECTION('ref_axis',(0.267631070012316,-0.823683738753064,-0.499918702268516));
#131218=DIRECTION('',(0.309016994374951,-0.951056516295152,-6.59767734033507E-15));
#131219=DIRECTION('center_axis',(-0.951056223677648,-0.309017894953224,
-1.64014399102986E-6));
#131220=DIRECTION('ref_axis',(0.267622092843757,-0.823656109146745,0.499969028327929));
#131221=DIRECTION('',(0.154510094588035,-0.475533174441031,0.866022419268943));
#131222=DIRECTION('',(0.309016994374951,-0.951056516295152,-6.59767734033507E-15));
#131223=DIRECTION('center_axis',(0.951056516295152,0.309016994374951,2.29177897539325E-15));
#131224=DIRECTION('ref_axis',(1.84331724214208E-16,6.84903784078409E-15,
-1.));
#131225=DIRECTION('center_axis',(-0.95105651629515,-0.309016994374958,-7.85678251079127E-15));
#131226=DIRECTION('ref_axis',(0.270281584632399,-0.831841183424754,0.484755722572828));
#131227=DIRECTION('',(-0.163755578933429,0.50398784940401,-0.848045021223106));
#131228=DIRECTION('',(0.309016994374951,-0.951056516295152,-6.45686043344516E-15));
#131229=DIRECTION('',(-0.16375574094135,0.503988348013116,0.848044693619245));
#131230=DIRECTION('center_axis',(-0.951056516295163,-0.30901699437492,-6.57488491631666E-14));
#131231=DIRECTION('ref_axis',(0.270282164140199,-0.831842966966367,-0.484752338886862));
#131232=DIRECTION('',(-0.309016994374951,0.951056516295152,6.59767734033507E-15));
#131233=DIRECTION('',(-0.15451009458806,0.475533174441019,-0.866022419268945));
#131234=DIRECTION('center_axis',(0.951056808949647,0.309016093671226,-1.64037043810308E-6));
#131235=DIRECTION('ref_axis',(0.267631101743103,-0.823683836411159,0.499918524376491));
#131236=DIRECTION('',(-0.309016994374951,0.951056516295152,6.59767734033507E-15));
#131237=DIRECTION('center_axis',(0.951056223742945,0.309017894752262,-1.6397776367882E-6));
#131238=DIRECTION('ref_axis',(0.267622060023681,-0.823656008137699,-0.499969212299469));
#131239=DIRECTION('',(-0.154510046201599,0.475533025522804,0.866022509672762));
#131240=DIRECTION('',(-0.309016994374951,0.951056516295152,6.59767734033507E-15));
#131241=DIRECTION('center_axis',(-1.98092302886631E-16,-6.85432003203771E-15,
1.));
#131242=DIRECTION('ref_axis',(-1.,1.38327115779427E-30,-1.98092302886631E-16));
#131243=DIRECTION('',(-0.406736643075804,0.913545457642599,6.18116153220146E-15));
#131244=DIRECTION('center_axis',(1.98092302886631E-16,6.85432003203771E-15,
-1.));
#131245=DIRECTION('ref_axis',(-1.,1.55513534684527E-30,-1.98092302886631E-16));
#131246=DIRECTION('',(0.406736643075804,-0.913545457642599,-6.18116153220146E-15));
#131247=DIRECTION('center_axis',(-1.98092302886631E-16,-6.85432003203771E-15,
1.));
#131248=DIRECTION('ref_axis',(-1.,1.25098969931104E-30,-1.98092302886631E-16));
#131249=DIRECTION('center_axis',(0.913545457642599,0.406736643075804,2.9688694438943E-15));
#131250=DIRECTION('ref_axis',(1.98092302886631E-16,6.85432003203771E-15,
-1.));
#131251=DIRECTION('center_axis',(0.913545457642599,0.406736643075804,-8.27029549119878E-16));
#131252=DIRECTION('ref_axis',(0.355752797173898,-0.799033864871854,-0.484752338922563));
#131253=DIRECTION('',(0.21553979738105,-0.484110311157671,-0.848044693619245));
#131254=DIRECTION('',(-0.406736643075804,0.913545457642599,6.18116153220146E-15));
#131255=DIRECTION('',(0.215539584141765,-0.484109832214438,0.848045021223109));
#131256=DIRECTION('center_axis',(0.913545457642593,0.406736643075818,2.34325092454483E-14));
#131257=DIRECTION('ref_axis',(0.355752034424608,-0.799032151708895,0.484755722543021));
#131258=DIRECTION('',(0.406736643075804,-0.913545457642599,-6.32197843909137E-15));
#131259=DIRECTION('',(0.20337036039278,-0.456777308164312,-0.866022509672743));
#131260=DIRECTION('center_axis',(-0.913545842753553,-0.406735778098031,
-1.6399888567167E-6));
#131261=DIRECTION('ref_axis',(0.352263354438044,-0.791196448576584,-0.499918702270538));
#131262=DIRECTION('',(0.406736643075804,-0.913545457642599,-6.32197843909137E-15));
#131263=DIRECTION('center_axis',(-0.91354507249199,-0.406737508133826,-1.6401440824322E-6));
#131264=DIRECTION('ref_axis',(0.352251538367414,-0.791169908698556,0.499969028328464));
#131265=DIRECTION('',(0.203370424080347,-0.456777451208943,0.866022419268948));
#131266=DIRECTION('',(0.406736643075804,-0.913545457642599,-6.32197843909137E-15));
#131267=DIRECTION('center_axis',(0.913545457642599,0.406736643075804,2.9688694438943E-15));
#131268=DIRECTION('ref_axis',(1.98092302886631E-16,6.85432003203771E-15,
-1.));
#131269=DIRECTION('center_axis',(-0.913545457642582,-0.406736643075842,
-7.44326764180192E-14));
#131270=DIRECTION('ref_axis',(0.355752034418312,-0.799032151694757,0.484755722570946));
#131271=DIRECTION('',(-0.21553958414177,0.484109832214447,-0.848045021223103));
#131272=DIRECTION('',(0.406736643075804,-0.913545457642599,-6.18116153220146E-15));
#131273=DIRECTION('',(-0.215539797381043,0.484110311157669,0.848044693619248));
#131274=DIRECTION('center_axis',(-0.913545457642587,-0.406736643075831,
3.94217418462606E-14));
#131275=DIRECTION('ref_axis',(0.355752797181838,-0.799033864889671,-0.484752338887366));
#131276=DIRECTION('',(-0.406736643075804,0.913545457642599,6.32197843909137E-15));
#131277=DIRECTION('',(-0.203370424080351,0.456777451208949,-0.866022419268944));
#131278=DIRECTION('center_axis',(0.913545842843072,0.406735777896966,-1.64037044955031E-6));
#131279=DIRECTION('ref_axis',(0.352263396204226,-0.791196542385554,0.499918524373531));
#131280=DIRECTION('',(-0.406736643075804,0.913545457642599,6.32197843909137E-15));
#131281=DIRECTION('center_axis',(0.913545072577991,0.406737507940666,-1.63977755898457E-6));
#131282=DIRECTION('ref_axis',(0.352251495169288,-0.791169811674637,-0.499969212297838));
#131283=DIRECTION('',(-0.203370360392795,0.456777308164266,0.866022509672764));
#131284=DIRECTION('',(-0.406736643075804,0.913545457642599,6.32197843909137E-15));
#131285=DIRECTION('center_axis',(-2.11225360334866E-16,-6.86101165903726E-15,
1.));
#131286=DIRECTION('ref_axis',(-1.,1.4749788077992E-30,-2.11225360334866E-16));
#131287=DIRECTION('',(-0.500000000000004,0.866025403784436,5.83619771222003E-15));
#131288=DIRECTION('center_axis',(2.11225360334866E-16,6.86101165903726E-15,
-1.));
#131289=DIRECTION('ref_axis',(-1.,1.55053706533811E-30,-2.11225360334866E-16));
#131290=DIRECTION('',(0.500000000000004,-0.866025403784436,-5.83619771222003E-15));
#131291=DIRECTION('center_axis',(-2.11225360334866E-16,-6.86101165903726E-15,
1.));
#131292=DIRECTION('ref_axis',(-1.,1.6579053986113E-30,-2.11225360334866E-16));
#131293=DIRECTION('center_axis',(0.866025403784436,0.500000000000004,3.61343235749217E-15));
#131294=DIRECTION('ref_axis',(2.11225360334867E-16,6.86101165903726E-15,
-1.));
#131295=DIRECTION('center_axis',(0.866025403784404,0.500000000000061,-7.33299533553082E-14));
#131296=DIRECTION('ref_axis',(0.437325728121665,-0.757470380563725,-0.484752338923188));
#131297=DIRECTION('',(0.264962354696018,-0.458928260426587,-0.84804469361925));
#131298=DIRECTION('',(-0.500000000000004,0.866025403784436,5.83619771222003E-15));
#131299=DIRECTION('',(0.264962092561705,-0.458927806396622,0.848045021223111));
#131300=DIRECTION('center_axis',(0.866025403784435,0.500000000000007,2.46730538525601E-14));
#131301=DIRECTION('ref_axis',(0.437324790476593,-0.757468756514882,0.484755722543223));
#131302=DIRECTION('',(0.500000000000004,-0.866025403784436,-5.97701461910994E-15));
#131303=DIRECTION('',(0.250002506357502,-0.433017043030757,-0.866022509672737));
#131304=DIRECTION('center_axis',(-0.866025877200505,-0.499999180015734,
-1.63998885809397E-6));
#131305=DIRECTION('ref_axis',(0.433036167836597,-0.750040644541319,-0.499918702272117));
#131306=DIRECTION('',(0.500000000000004,-0.866025403784436,-5.97701461910994E-15));
#131307=DIRECTION('center_axis',(-0.866024930320587,-0.50000082005986,-1.64014391649668E-6));
#131308=DIRECTION('ref_axis',(0.433021642321137,-0.750015485164071,0.499969028336364));
#131309=DIRECTION('',(0.250002584648427,-0.433017178634617,0.866022419268937));
#131310=DIRECTION('',(0.500000000000004,-0.866025403784436,-5.97701461910994E-15));
#131311=DIRECTION('center_axis',(0.866025403784436,0.500000000000004,3.61343235749217E-15));
#131312=DIRECTION('ref_axis',(2.11225360334867E-16,6.86101165903726E-15,
-1.));
#131313=DIRECTION('center_axis',(-0.866025403784421,-0.50000000000003,-5.320557980992E-14));
#131314=DIRECTION('ref_axis',(0.437324790468157,-0.757468756500253,0.484755722573692));
#131315=DIRECTION('',(-0.264962092561701,0.458927806396626,-0.84804502122311));
#131316=DIRECTION('',(0.500000000000004,-0.866025403784436,-5.83619771222003E-15));
#131317=DIRECTION('',(-0.264962354696035,0.45892826042661,0.848044693619233));
#131318=DIRECTION('center_axis',(-0.866025403784439,-0.5,-2.48108864766685E-14));
#131319=DIRECTION('ref_axis',(0.437325728131541,-0.75747038058086,-0.484752338887502));
#131320=DIRECTION('',(-0.500000000000004,0.866025403784436,5.97701461910994E-15));
#131321=DIRECTION('',(-0.250002584648417,0.433017178634595,-0.866022419268951));
#131322=DIRECTION('center_axis',(0.86602587731055,0.499999179825129,-1.64037040961549E-6));
#131323=DIRECTION('ref_axis',(0.433036219180504,-0.750040733472094,0.49991852437222));
#131324=DIRECTION('',(-0.500000000000004,0.866025403784436,5.97701461910994E-15));
#131325=DIRECTION('center_axis',(0.866024930426257,0.500000819876835,-1.6397775689687E-6));
#131326=DIRECTION('ref_axis',(0.433021589219912,-0.750015393190588,-0.499969212298748));
#131327=DIRECTION('',(-0.250002506357468,0.433017043030729,0.866022509672762));
#131328=DIRECTION('',(-0.500000000000004,0.866025403784436,5.97701461910994E-15));
#131329=DIRECTION('center_axis',(-2.23587008033243E-16,-6.86903940691702E-15,
1.));
#131330=DIRECTION('ref_axis',(-1.,1.56129973231167E-30,-2.23587008033243E-16));
#131331=DIRECTION('',(-0.587785252292477,0.809016994374945,5.42574846930092E-15));
#131332=DIRECTION('center_axis',(2.23587008033243E-16,6.86903940691702E-15,
-1.));
#131333=DIRECTION('ref_axis',(-1.,2.1582735598713E-13,-2.2358700803176E-16));
#131334=DIRECTION('',(0.587785252292477,-0.809016994374945,-5.42574846930092E-15));
#131335=DIRECTION('center_axis',(-2.23587008033243E-16,-6.86903940691702E-15,
1.));
#131336=DIRECTION('ref_axis',(-1.,1.69233669110578E-30,-2.23587008033243E-16));
#131337=DIRECTION('center_axis',(0.809016994374945,0.587785252292477,4.21840575002203E-15));
#131338=DIRECTION('ref_axis',(2.23587008033243E-16,6.86903940691702E-15,
-1.));
#131339=DIRECTION('center_axis',(0.809016994374947,0.587785252292474,1.54378849169051E-14));
#131340=DIRECTION('ref_axis',(0.514107226876102,-0.707607892255824,-0.484752338922705));
#131341=DIRECTION('',(0.311481929006018,-0.428718095637362,-0.848044693619248));
#131342=DIRECTION('',(-0.587785252292477,0.809016994374945,5.42574846930092E-15));
#131343=DIRECTION('',(0.311481620848644,-0.428717671495135,0.848045021223102));
#131344=DIRECTION('center_axis',(0.809016994374931,0.587785252292496,3.47352489991332E-14));
#131345=DIRECTION('ref_axis',(0.514106124607984,-0.707606375113916,0.484755722543533));
#131346=DIRECTION('',(0.587785252292477,-0.809016994374945,-5.56656537619083E-15));
#131347=DIRECTION('',(0.29389557254618,-0.404512552559093,-0.866022509672745));
#131348=DIRECTION('center_axis',(-0.809017550909332,-0.587784486285558,
-1.63998894398804E-6));
#131349=DIRECTION('ref_axis',(0.509064546361577,-0.70066723824859,-0.499918702273455));
#131350=DIRECTION('',(0.587785252292477,-0.809016994374945,-5.56656537619083E-15));
#131351=DIRECTION('center_axis',(-0.80901643778517,-0.587786018369528,-1.64014399843157E-6));
#131352=DIRECTION('ref_axis',(0.509047470549497,-0.700643735029776,0.49996902833144));
#131353=DIRECTION('',(0.293895664582661,-0.404512679236465,0.866022419268955));
#131354=DIRECTION('',(0.587785252292477,-0.809016994374945,-5.56656537619083E-15));
#131355=DIRECTION('center_axis',(0.809016994374945,0.587785252292477,4.21840575002203E-15));
#131356=DIRECTION('ref_axis',(2.23587008033243E-16,6.86903940691702E-15,
-1.));
#131357=DIRECTION('center_axis',(-0.809016994374898,-0.587785252292541,
-1.25984196751993E-13));
#131358=DIRECTION('ref_axis',(0.514106124597603,-0.70760637509962,0.484755722575412));
#131359=DIRECTION('',(-0.311481620848633,0.428717671495124,-0.848045021223112));
#131360=DIRECTION('',(0.587785252292477,-0.809016994374945,-5.42574846930092E-15));
#131361=DIRECTION('',(-0.311481929006027,0.428718095637352,0.84804469361925));
#131362=DIRECTION('center_axis',(-0.80901699437497,-0.587785252292442,-5.73407154127436E-14));
#131363=DIRECTION('ref_axis',(0.514107226887343,-0.707607892271321,-0.484752338888164));
#131364=DIRECTION('',(-0.587785252292477,0.809016994374945,5.56656537619083E-15));
#131365=DIRECTION('',(-0.293895664582678,0.404512679236454,-0.866022419268954));
#131366=DIRECTION('center_axis',(0.809017551038645,0.587784486107572,-1.64037042941065E-6));
#131367=DIRECTION('ref_axis',(0.509064606719126,-0.700667321323996,0.49991852437628));
#131368=DIRECTION('',(-0.587785252292477,0.809016994374945,5.56656537619083E-15));
#131369=DIRECTION('center_axis',(0.80901643790939,0.587786018198556,-1.63977758015677E-6));
#131370=DIRECTION('ref_axis',(0.509047408125087,-0.700643649110335,-0.499969212294602));
#131371=DIRECTION('',(-0.293895572546205,0.40451255255908,0.866022509672743));
#131372=DIRECTION('',(-0.587785252292477,0.809016994374945,5.56656537619083E-15));
#131373=DIRECTION('center_axis',(-2.35041809182736E-16,-6.8783153219913E-15,
1.));
#131374=DIRECTION('ref_axis',(-1.,1.6412881812189E-30,-2.35041809182736E-16));
#131375=DIRECTION('',(-0.669130606358862,0.743144825477391,4.95431077124156E-15));
#131376=DIRECTION('center_axis',(2.35041809182736E-16,6.8783153219913E-15,
-1.));
#131377=DIRECTION('ref_axis',(-1.,1.57191309186665E-30,-2.35041809182736E-16));
#131378=DIRECTION('',(0.669130606358862,-0.743144825477391,-4.95431077124156E-15));
#131379=DIRECTION('center_axis',(-2.35041809182736E-16,-6.8783153219913E-15,
1.));
#131380=DIRECTION('ref_axis',(-1.,1.6700863880665E-30,-2.35041809182736E-16));
#131381=DIRECTION('center_axis',(0.743144825477391,0.669130606358862,4.77716140639648E-15));
#131382=DIRECTION('ref_axis',(2.35041809182736E-16,6.8783153219913E-15,
-1.));
#131383=DIRECTION('center_axis',(0.743144825477429,0.669130606358819,1.07238164869218E-13));
#131384=DIRECTION('ref_axis',(0.585256059269502,-0.649992703804315,-0.484752338921114));
#131385=DIRECTION('',(0.354588842120036,-0.393810805677314,-0.848044693619244));
#131386=DIRECTION('',(-0.669130606358862,0.743144825477391,4.95431077124156E-15));
#131387=DIRECTION('',(0.354588491315835,-0.393810416069778,0.848045021223112));
#131388=DIRECTION('center_axis',(0.743144825477371,0.669130606358884,3.96974274275828E-14));
#131389=DIRECTION('ref_axis',(0.585254804454859,-0.649991310191462,0.484755722542903));
#131390=DIRECTION('',(0.669130606358862,-0.743144825477391,-5.09512767813147E-15));
#131391=DIRECTION('',(0.334568657340445,-0.371576137911944,-0.866022509672731));
#131392=DIRECTION('center_axis',(-0.743145459032541,-0.669129902721903,
-1.63998892591404E-6));
#131393=DIRECTION('ref_axis',(0.579515507190066,-0.643617175072043,-0.499918702269203));
#131394=DIRECTION('',(0.669130606358862,-0.743144825477391,-5.09512767813147E-15));
#131395=DIRECTION('center_axis',(-0.743144191859853,-0.669131310059748,
-1.64014385074246E-6));
#131396=DIRECTION('ref_axis',(0.579496068163196,-0.64359558551187,0.499969028333786));
#131397=DIRECTION('',(0.334568762114132,-0.371576254274909,0.866022419268951));
#131398=DIRECTION('',(0.669130606358862,-0.743144825477391,-5.09512767813147E-15));
#131399=DIRECTION('center_axis',(0.743144825477391,0.669130606358862,4.77716140639648E-15));
#131400=DIRECTION('ref_axis',(2.35041809182736E-16,6.8783153219913E-15,
-1.));
#131401=DIRECTION('center_axis',(-0.743144825477371,-0.669130606358884,
-6.75407619348696E-14));
#131402=DIRECTION('ref_axis',(0.585254804443369,-0.649991310178721,0.484755722573859));
#131403=DIRECTION('',(-0.354588491315836,0.39381041606978,-0.848045021223111));
#131404=DIRECTION('',(0.669130606358862,-0.743144825477391,-4.95431077124156E-15));
#131405=DIRECTION('',(-0.354588842120062,0.393810805677293,0.848044693619243));
#131406=DIRECTION('center_axis',(-0.743144825477435,-0.669130606358813,
-9.70381337754059E-14));
#131407=DIRECTION('ref_axis',(0.585256059282122,-0.649992703818349,-0.484752338887059));
#131408=DIRECTION('',(-0.669130606358862,0.743144825477391,5.09512767813147E-15));
#131409=DIRECTION('',(-0.334568762114163,0.371576254274904,-0.86602241926894));
#131410=DIRECTION('center_axis',(0.743145459179803,0.669129902558351,-1.64037053045256E-6));
#131411=DIRECTION('ref_axis',(0.579515575900153,-0.643617251382659,0.499918524373468));
#131412=DIRECTION('',(-0.669130606358862,0.743144825477391,5.09512767813147E-15));
#131413=DIRECTION('center_axis',(0.743144192001209,0.669131309902759,-1.63977761596072E-6));
#131414=DIRECTION('ref_axis',(0.579495997099647,-0.643595506588175,-0.499969212297114));
#131415=DIRECTION('',(-0.334568657340465,0.371576137911926,0.866022509672731));
#131416=DIRECTION('',(-0.669130606358862,0.743144825477391,5.09512767813147E-15));
#131417=DIRECTION('center_axis',(-2.4546426258488E-16,-6.88873777539344E-15,
1.));
#131418=DIRECTION('ref_axis',(-1.,1.714067784336E-30,-2.4546426258488E-16));
#131419=DIRECTION('',(-0.743144825477398,0.669130606358854,4.42704978811658E-15));
#131420=DIRECTION('center_axis',(2.4546426258488E-16,6.88873777539344E-15,
-1.));
#131421=DIRECTION('ref_axis',(-1.,1.54864157893911E-30,-2.4546426258488E-16));
#131422=DIRECTION('',(0.743144825477398,-0.669130606358854,-4.42704978811658E-15));
#131423=DIRECTION('center_axis',(-2.4546426258488E-16,-6.88873777539344E-15,
1.));
#131424=DIRECTION('ref_axis',(-1.,1.6912719677966E-30,-2.4546426258488E-16));
#131425=DIRECTION('center_axis',(0.669130606358854,0.743144825477398,5.28357748271717E-15));
#131426=DIRECTION('ref_axis',(2.4546426258488E-16,6.88873777539344E-15,
-1.));
#131427=DIRECTION('center_axis',(0.669130606358848,0.743144825477403,-9.09732504031885E-15));
#131428=DIRECTION('ref_axis',(0.649992703803272,-0.585256059268544,-0.484752338923668));
#131429=DIRECTION('',(0.393810805677323,-0.354588842120038,-0.848044693619239));
#131430=DIRECTION('',(-0.743144825477398,0.669130606358854,4.42704978811658E-15));
#131431=DIRECTION('',(0.393810416069788,-0.354588491315845,0.848045021223103));
#131432=DIRECTION('center_axis',(0.669130606358885,0.74314482547737,-4.46596058560287E-14));
#131433=DIRECTION('ref_axis',(0.649991310190434,-0.585254804453932,0.4847557225454));
#131434=DIRECTION('',(0.743144825477398,-0.669130606358854,-4.56786669500649E-15));
#131435=DIRECTION('',(0.371576137911948,-0.334568657340484,-0.866022509672714));
#131436=DIRECTION('center_axis',(-0.669131309993376,-0.743144191919616,
-1.63998892143862E-6));
#131437=DIRECTION('ref_axis',(0.643617174848185,-0.579515507437152,-0.499918702270981));
#131438=DIRECTION('',(0.743144825477398,-0.669130606358854,-4.56786669500649E-15));
#131439=DIRECTION('center_axis',(-0.669129902655549,-0.743145459092287,
-1.64014392097245E-6));
#131440=DIRECTION('ref_axis',(0.643595585587833,-0.579496068079466,0.499969028333048));
#131441=DIRECTION('',(0.371576254274914,-0.334568762114171,0.866022419268933));
#131442=DIRECTION('',(0.743144825477398,-0.669130606358854,-4.56786669500649E-15));
#131443=DIRECTION('center_axis',(0.669130606358854,0.743144825477398,5.28357748271717E-15));
#131444=DIRECTION('ref_axis',(2.4546426258488E-16,6.88873777539344E-15,
-1.));
#131445=DIRECTION('center_axis',(-0.669130606358856,-0.743144825477396,
2.3156832663386E-14));
#131446=DIRECTION('ref_axis',(0.649991310178511,-0.585254804443164,0.484755722574387));
#131447=DIRECTION('',(-0.393810416069763,0.35458849131586,-0.848045021223108));
#131448=DIRECTION('',(0.743144825477398,-0.669130606358854,-4.42704978811658E-15));
#131449=DIRECTION('',(-0.393810805677305,0.354588842120013,0.848044693619257));
#131450=DIRECTION('center_axis',(-0.669130606358852,-0.7431448254774,-1.18540902055189E-14));
#131451=DIRECTION('ref_axis',(0.649992703818265,-0.585256059282037,-0.484752338887274));
#131452=DIRECTION('',(-0.743144825477398,0.669130606358854,4.56786669500649E-15));
#131453=DIRECTION('',(-0.3715762542749,0.334568762114124,-0.866022419268957));
#131454=DIRECTION('center_axis',(0.669131310156853,0.743144191772419,-1.64037024591789E-6));
#131455=DIRECTION('ref_axis',(0.643617251157576,-0.579515576146809,0.499918524377321));
#131456=DIRECTION('',(-0.743144825477398,0.669130606358854,4.56786669500649E-15));
#131457=DIRECTION('center_axis',(0.669129902812627,0.743145458950854,-1.63977753884496E-6));
#131458=DIRECTION('ref_axis',(0.643595506662832,-0.57949599701545,-0.4999692122986));
#131459=DIRECTION('',(-0.371576137911895,0.334568657340398,0.86602250967277));
#131460=DIRECTION('',(-0.743144825477398,0.669130606358854,4.56786669500649E-15));
#131461=DIRECTION('center_axis',(-2.54740177659163E-16,-6.90019257654294E-15,
1.));
#131462=DIRECTION('ref_axis',(-1.,1.77884115310111E-30,-2.54740177659163E-16));
#131463=DIRECTION('',(-0.80901699437495,0.587785252292469,3.84974230159355E-15));
#131464=DIRECTION('center_axis',(2.54740177659163E-16,6.90019257654294E-15,
-1.));
#131465=DIRECTION('ref_axis',(-1.,-1.4388490399142E-13,-2.54740177660156E-16));
#131466=DIRECTION('',(0.80901699437495,-0.587785252292469,-3.84974230159355E-15));
#131467=DIRECTION('center_axis',(-2.54740177659163E-16,-6.90019257654294E-15,
1.));
#131468=DIRECTION('ref_axis',(-1.,1.65392111781157E-30,-2.54740177659163E-16));
#131469=DIRECTION('center_axis',(0.587785252292469,0.80901699437495,5.73210557847753E-15));
#131470=DIRECTION('ref_axis',(2.54740177659164E-16,6.90019257654294E-15,
-1.));
#131471=DIRECTION('center_axis',(0.587785252292465,0.809016994374953,-2.72919751209577E-14));
#131472=DIRECTION('ref_axis',(0.707607892255939,-0.51410722687618,-0.484752338922456));
#131473=DIRECTION('',(0.428718095637376,-0.311481929006005,-0.848044693619245));
#131474=DIRECTION('',(-0.80901699437495,0.587785252292469,3.84974230159355E-15));
#131475=DIRECTION('',(0.428717671495123,-0.311481620848632,0.848045021223112));
#131476=DIRECTION('center_axis',(0.587785252292479,0.809016994374943,-1.0613548305292E-14));
#131477=DIRECTION('ref_axis',(0.707606375113318,-0.514106124607541,0.484755722544878));
#131478=DIRECTION('',(0.80901699437495,-0.587785252292469,-3.99055920848346E-15));
#131479=DIRECTION('',(0.40451255255906,-0.293895572546216,-0.866022509672749));
#131480=DIRECTION('center_axis',(-0.587786018297275,-0.809016437837666,
-1.63998894467645E-6));
#131481=DIRECTION('ref_axis',(0.700667238054855,-0.509064546632989,-0.49991870226861));
#131482=DIRECTION('',(0.80901699437495,-0.587785252292469,-3.99055920848346E-15));
#131483=DIRECTION('center_axis',(-0.587784486213231,-0.80901755096188,-1.64014414198988E-6));
#131484=DIRECTION('ref_axis',(0.700643735095494,-0.509047470457538,0.499969028332974));
#131485=DIRECTION('',(0.404512679236436,-0.293895664582665,0.866022419268967));
#131486=DIRECTION('',(0.80901699437495,-0.587785252292469,-3.99055920848346E-15));
#131487=DIRECTION('center_axis',(0.587785252292469,0.80901699437495,5.73210557847753E-15));
#131488=DIRECTION('ref_axis',(2.54740177659164E-16,6.90019257654294E-15,
-1.));
#131489=DIRECTION('center_axis',(-0.58778525229251,-0.809016994374921,1.17438222792872E-13));
#131490=DIRECTION('ref_axis',(0.707606375100373,-0.514106124598113,0.484755722573772));
#131491=DIRECTION('',(-0.428717671495135,0.311481620848657,-0.848045021223097));
#131492=DIRECTION('',(0.80901699437495,-0.587785252292469,-3.84974230159355E-15));
#131493=DIRECTION('',(-0.428718095637387,0.311481929006017,0.848044693619235));
#131494=DIRECTION('center_axis',(-0.587785252292488,-0.809016994374937,
-2.37081804110383E-14));
#131495=DIRECTION('ref_axis',(0.707607892271278,-0.514107226887325,-0.484752338888244));
#131496=DIRECTION('',(-0.80901699437495,0.587785252292469,3.99055920848346E-15));
#131497=DIRECTION('',(-0.404512679236475,0.293895664582667,-0.866022419268948));
#131498=DIRECTION('center_axis',(0.58778601847531,0.809016437708315,-1.64037048156678E-6));
#131499=DIRECTION('ref_axis',(0.700667321127577,-0.509064606989155,0.499918524376605));
#131500=DIRECTION('',(-0.80901699437495,0.587785252292469,3.99055920848346E-15));
#131501=DIRECTION('center_axis',(0.587784486384294,0.809017550837597,-1.63977761045217E-6));
#131502=DIRECTION('ref_axis',(0.700643649175082,-0.509047408033036,-0.49996921229759));
#131503=DIRECTION('',(-0.404512552559104,0.293895572546197,0.866022509672734));
#131504=DIRECTION('',(-0.80901699437495,0.587785252292469,3.99055920848346E-15));
#131505=DIRECTION('center_axis',(-2.62767925538921E-16,-6.91255422424131E-15,
1.));
#131506=DIRECTION('ref_axis',(-1.,1.83489861693133E-30,-2.62767925538921E-16));
#131507=DIRECTION('',(-0.866025403784441,0.499999999999995,3.22871341330418E-15));
#131508=DIRECTION('center_axis',(2.62767925538921E-16,6.91255422424131E-15,
-1.));
#131509=DIRECTION('ref_axis',(-1.,-1.19904086659517E-13,-2.6276792553975E-16));
#131510=DIRECTION('',(0.866025403784441,-0.499999999999995,-3.22871341330418E-15));
#131511=DIRECTION('center_axis',(-2.62767925538921E-16,-6.91255422424131E-15,
1.));
#131512=DIRECTION('ref_axis',(-1.,1.65859733677587E-30,-2.62767925538921E-16));
#131513=DIRECTION('center_axis',(0.499999999999995,0.866025403784442,6.11783152599989E-15));
#131514=DIRECTION('ref_axis',(2.62767925538921E-16,6.91255422424131E-15,
-1.));
#131515=DIRECTION('center_axis',(0.499999999999996,0.866025403784441,3.41838880302928E-14));
#131516=DIRECTION('ref_axis',(0.757470380564982,-0.437325728122336,-0.484752338920618));
#131517=DIRECTION('',(0.458928260426605,-0.264962354696014,-0.848044693619242));
#131518=DIRECTION('',(-0.866025403784442,0.499999999999995,3.22871341330418E-15));
#131519=DIRECTION('',(0.458927806396632,-0.264962092561704,0.848045021223106));
#131520=DIRECTION('center_axis',(0.499999999999982,0.866025403784449,3.4597410709456E-14));
#131521=DIRECTION('ref_axis',(0.757468756515396,-0.437324790476894,0.484755722542148));
#131522=DIRECTION('',(0.866025403784442,-0.499999999999995,-3.36953032019409E-15));
#131523=DIRECTION('',(0.43301704303075,-0.250002506357463,-0.866022509672752));
#131524=DIRECTION('center_axis',(-0.500000819982456,-0.866024930365277,
-1.63998877357693E-6));
#131525=DIRECTION('ref_axis',(0.75004064437554,-0.433036168125902,-0.49991870227024));
#131526=DIRECTION('',(0.866025403784442,-0.499999999999995,-3.36953032019409E-15));
#131527=DIRECTION('center_axis',(-0.4999991799383,-0.866025877245211,-1.64014404112045E-6));
#131528=DIRECTION('ref_axis',(0.75001548522118,-0.433021642223581,0.499969028335187));
#131529=DIRECTION('',(0.433017178634605,-0.250002584648423,0.866022419268944));
#131530=DIRECTION('',(0.866025403784442,-0.499999999999995,-3.36953032019409E-15));
#131531=DIRECTION('center_axis',(0.499999999999995,0.866025403784442,6.11783152599989E-15));
#131532=DIRECTION('ref_axis',(2.62767925538921E-16,6.91255422424131E-15,
-1.));
#131533=DIRECTION('center_axis',(-0.500000000000014,-0.866025403784431,
5.2378550071941E-14));
#131534=DIRECTION('ref_axis',(0.757468756500337,-0.437324790468187,0.484755722573535));
#131535=DIRECTION('',(-0.458927806396645,0.264962092561697,-0.848045021223101));
#131536=DIRECTION('',(0.866025403784442,-0.499999999999995,-3.22871341330418E-15));
#131537=DIRECTION('',(-0.458928260426594,0.264962354696015,0.848044693619248));
#131538=DIRECTION('center_axis',(-0.5,-0.866025403784439,-4.50731104326131E-14));
#131539=DIRECTION('ref_axis',(0.757470380581421,-0.437325728131826,-0.484752338886368));
#131540=DIRECTION('',(-0.866025403784442,0.499999999999995,3.36953032019409E-15));
#131541=DIRECTION('',(-0.433017178634586,0.250002584648412,-0.866022419268957));
#131542=DIRECTION('center_axis',(0.500000820173086,0.866024930255215,-1.64037043715635E-6));
#131543=DIRECTION('ref_axis',(0.750040733300453,-0.433036219466989,0.499918524381581));
#131544=DIRECTION('',(-0.866025403784442,0.499999999999995,3.36953032019409E-15));
#131545=DIRECTION('center_axis',(0.499999180121306,0.866025877139554,-1.63977767534645E-6));
#131546=DIRECTION('ref_axis',(0.750015393247303,-0.433021589122715,-0.499969212297849));
#131547=DIRECTION('',(-0.433017043030757,0.250002506357464,0.866022509672748));
#131548=DIRECTION('',(-0.866025403784442,0.499999999999995,3.36953032019409E-15));
#131549=DIRECTION('center_axis',(-2.6945955253847E-16,-6.92568728168955E-15,
1.));
#131550=DIRECTION('ref_axis',(-1.,1.88162599852217E-30,-2.6945955253847E-16));
#131551=DIRECTION('',(-0.913545457642603,0.406736643075795,2.57076724570721E-15));
#131552=DIRECTION('center_axis',(2.6945955253847E-16,6.92568728168955E-15,
-1.));
#131553=DIRECTION('ref_axis',(-1.,4.79616346638067E-14,-2.69459552538137E-16));
#131554=DIRECTION('',(0.913545457642603,-0.406736643075795,-2.57076724570721E-15));
#131555=DIRECTION('center_axis',(-2.6945955253847E-16,-6.92568728168955E-15,
1.));
#131556=DIRECTION('ref_axis',(-1.,2.07166276942212E-30,-2.6945955253847E-16));
#131557=DIRECTION('center_axis',(0.406736643075795,0.913545457642603,6.43652923108484E-15));
#131558=DIRECTION('ref_axis',(2.6945955253847E-16,6.92568728168955E-15,
-1.));
#131559=DIRECTION('center_axis',(0.406736643075755,0.913545457642621,-7.60867185190334E-14));
#131560=DIRECTION('ref_axis',(0.799033864872018,-0.355752797173961,-0.484752338922246));
#131561=DIRECTION('',(0.484110311157685,-0.215539797381024,-0.848044693619243));
#131562=DIRECTION('',(-0.913545457642603,0.406736643075795,2.5707672457072E-15));
#131563=DIRECTION('',(0.484109832214428,-0.21553958414178,0.848045021223111));
#131564=DIRECTION('center_axis',(0.406736643075769,0.913545457642615,5.37569329748505E-14));
#131565=DIRECTION('ref_axis',(0.799032151707873,-0.355752034424143,0.484755722545047));
#131566=DIRECTION('',(0.913545457642603,-0.406736643075795,-2.71158415259712E-15));
#131567=DIRECTION('',(0.456777308164332,-0.203370360392738,-0.866022509672742));
#131568=DIRECTION('center_axis',(-0.406737508052088,-0.913545072528383,
-1.63998878579854E-6));
#131569=DIRECTION('ref_axis',(0.791196448440653,-0.352263354742521,-0.499918702271121));
#131570=DIRECTION('',(0.913545457642603,-0.406736643075795,-2.71158415259712E-15));
#131571=DIRECTION('center_axis',(-0.406735778016336,-0.913545842789926,
-1.6401440662521E-6));
#131572=DIRECTION('ref_axis',(0.791169908742451,-0.352251538263208,0.499969028332421));
#131573=DIRECTION('',(0.456777451208934,-0.203370424080325,0.866022419268958));
#131574=DIRECTION('',(0.913545457642603,-0.406736643075795,-2.71158415259712E-15));
#131575=DIRECTION('center_axis',(0.406736643075795,0.913545457642603,6.43652923108484E-15));
#131576=DIRECTION('ref_axis',(2.6945955253847E-16,6.92568728168955E-15,
-1.));
#131577=DIRECTION('center_axis',(-0.406736643075775,-0.913545457642612,
-2.39838624013607E-14));
#131578=DIRECTION('ref_axis',(0.799032151693213,-0.355752034417607,0.484755722574007));
#131579=DIRECTION('',(-0.48410983221445,0.215539584141779,-0.848045021223099));
#131580=DIRECTION('',(0.913545457642603,-0.406736643075795,-2.5707672457072E-15));
#131581=DIRECTION('',(-0.484110311157682,0.21553979738103,0.848044693619243));
#131582=DIRECTION('center_axis',(-0.40673664307581,-0.913545457642596,-1.53000466606117E-14));
#131583=DIRECTION('ref_axis',(0.799033864890076,-0.35575279718201,-0.484752338886573));
#131584=DIRECTION('',(-0.913545457642603,0.406736643075795,2.71158415259712E-15));
#131585=DIRECTION('',(-0.456777451208944,0.203370424080347,-0.866022419268947));
#131586=DIRECTION('center_axis',(0.406737508253247,0.91354507243882,-1.6403705445672E-6));
#131587=DIRECTION('ref_axis',(0.791196542249301,-0.352263396509092,0.49991852437435));
#131588=DIRECTION('',(-0.913545457642603,0.406736643075795,2.71158415259712E-15));
#131589=DIRECTION('center_axis',(0.406735778209435,0.913545842703954,-1.63977762938691E-6));
#131590=DIRECTION('ref_axis',(0.791169811721884,-0.352251495067145,-0.499969212295037));
#131591=DIRECTION('',(-0.456777308164335,0.203370360392759,0.866022509672736));
#131592=DIRECTION('',(-0.913545457642603,0.406736643075795,2.71158415259712E-15));
#131593=DIRECTION('center_axis',(-2.74741743792088E-16,-6.93944786036197E-15,
1.));
#131594=DIRECTION('ref_axis',(-1.,1.91851134290259E-30,-2.74741743792088E-16));
#131595=DIRECTION('',(-0.951056516295155,0.309016994374942,1.88311239469892E-15));
#131596=DIRECTION('center_axis',(2.74741743792088E-16,6.93944786036197E-15,
-1.));
#131597=DIRECTION('ref_axis',(-1.,3.5527136788005E-14,-2.74741743791841E-16));
#131598=DIRECTION('',(0.951056516295155,-0.309016994374942,-1.88311239469892E-15));
#131599=DIRECTION('center_axis',(-2.74741743792088E-16,-6.93944786036197E-15,
1.));
#131600=DIRECTION('ref_axis',(-1.,2.10828553426994E-30,-2.74741743792088E-16));
#131601=DIRECTION('center_axis',(0.309016994374942,0.951056516295155,6.68470697498369E-15));
#131602=DIRECTION('ref_axis',(2.74741743792088E-16,6.93944786036197E-15,
-1.));
#131603=DIRECTION('center_axis',(0.309016994374954,0.951056516295151,2.34325038917348E-14));
#131604=DIRECTION('ref_axis',(0.831842966947239,-0.270282164133971,-0.484752338923158));
#131605=DIRECTION('',(0.503988348013129,-0.163755740941344,-0.848044693619239));
#131606=DIRECTION('',(-0.951056516295155,0.309016994374942,1.88311239469892E-15));
#131607=DIRECTION('',(0.503987849404003,-0.163755578933424,0.848045021223111));
#131608=DIRECTION('center_axis',(0.309016994374937,0.951056516295157,9.51084198785806E-15));
#131609=DIRECTION('ref_axis',(0.83184118343951,-0.270281584637182,0.484755722544839));
#131610=DIRECTION('',(0.951056516295155,-0.309016994374942,-2.02392930158883E-15));
#131611=DIRECTION('',(0.475533025522856,-0.154510046201578,-0.866022509672736));
#131612=DIRECTION('center_axis',(-0.309017894868182,-0.95105622370528,-1.63998878906873E-6));
#131613=DIRECTION('ref_axis',(0.823683738647416,-0.26763107032859,-0.499918702273269));
#131614=DIRECTION('',(0.951056516295155,-0.309016994374942,-2.02392930158883E-15));
#131615=DIRECTION('center_axis',(-0.309016093795536,-0.951056808909257,
-1.64014398896477E-6));
#131616=DIRECTION('ref_axis',(0.823656109179533,-0.267622092735545,0.499969028331835));
#131617=DIRECTION('',(0.475533174441014,-0.154510094588067,0.866022419268946));
#131618=DIRECTION('',(0.951056516295155,-0.309016994374942,-2.02392930158883E-15));
#131619=DIRECTION('center_axis',(0.309016994374942,0.951056516295155,6.68470697498369E-15));
#131620=DIRECTION('ref_axis',(2.74741743792088E-16,6.93944786036197E-15,
-1.));
#131621=DIRECTION('center_axis',(-0.309016994374951,-0.951056516295152,
3.72163382090124E-15));
#131622=DIRECTION('ref_axis',(0.831841183423651,-0.270281584632036,0.484755722574922));
#131623=DIRECTION('',(-0.503987849404007,0.163755578933431,-0.848045021223107));
#131624=DIRECTION('',(0.951056516295155,-0.309016994374942,-1.88311239469892E-15));
#131625=DIRECTION('',(-0.503988348013115,0.163755740941334,0.848044693619249));
#131626=DIRECTION('center_axis',(-0.309016994374943,-0.951056516295155,
-1.51622084024086E-14));
#131627=DIRECTION('ref_axis',(0.831842966966906,-0.270282164140354,-0.48475233888585));
#131628=DIRECTION('',(-0.951056516295155,0.309016994374942,2.02392930158883E-15));
#131629=DIRECTION('',(-0.475533174441028,0.154510094588078,-0.866022419268937));
#131630=DIRECTION('center_axis',(0.30901789507753,0.951056223637258,-1.64037039627468E-6));
#131631=DIRECTION('ref_axis',(0.823683836309039,-0.267631102061046,0.499918524374537));
#131632=DIRECTION('',(-0.951056516295155,0.309016994374942,2.02392930158883E-15));
#131633=DIRECTION('center_axis',(0.309016093996548,0.951056808843945,-1.63977760305072E-6));
#131634=DIRECTION('ref_axis',(0.823656008173282,-0.267622059916903,-0.499969212298005));
#131635=DIRECTION('',(-0.475533025522834,0.154510046201571,0.86602250967275));
#131636=DIRECTION('',(-0.951056516295155,0.309016994374942,2.02392930158883E-15));
#131637=DIRECTION('center_axis',(-2.78556626507032E-16,-6.95368519647906E-15,
1.));
#131638=DIRECTION('ref_axis',(-1.,1.9451505265208E-30,-2.78556626507032E-16));
#131639=DIRECTION('',(-0.978147600733807,0.207911690817753,1.17328295072798E-15));
#131640=DIRECTION('center_axis',(2.78556626507032E-16,6.95368519647906E-15,
-1.));
#131641=DIRECTION('ref_axis',(-1.,1.15463194561016E-14,-2.78556626506952E-16));
#131642=DIRECTION('',(0.978147600733807,-0.207911690817753,-1.17328295072798E-15));
#131643=DIRECTION('center_axis',(-2.78556626507032E-16,-6.95368519647906E-15,
1.));
#131644=DIRECTION('ref_axis',(-1.,2.08376587424813E-30,-2.78556626507032E-16));
#131645=DIRECTION('center_axis',(0.207911690817753,0.978147600733807,6.85964567039975E-15));
#131646=DIRECTION('ref_axis',(2.78556626507032E-16,6.95368519647906E-15,
-1.));
#131647=DIRECTION('center_axis',(0.207911690817757,0.978147600733806,1.02000311058128E-14));
#131648=DIRECTION('ref_axis',(0.855538223403065,-0.181850263143827,-0.484752338922514));
#131649=DIRECTION('',(0.518344583061388,-0.110177542335806,-0.848044693619244));
#131650=DIRECTION('',(-0.978147600733807,0.207911690817753,1.17328295072798E-15));
#131651=DIRECTION('',(0.518344070249267,-0.110177433334231,0.848045021223109));
#131652=DIRECTION('center_axis',(0.207911690817748,0.978147600733808,1.44730204163055E-14));
#131653=DIRECTION('ref_axis',(0.855536389092135,-0.181849873249007,0.484755722543334));
#131654=DIRECTION('',(0.978147600733807,-0.207911690817753,-1.3140998576179E-15));
#131655=DIRECTION('',(0.489078703542099,-0.103956887610937,-0.866022509672714));
#131656=DIRECTION('center_axis',(-0.207912616961996,-0.978147403873938,
-1.63998882728223E-6));
#131657=DIRECTION('ref_axis',(0.847146577450082,-0.180066563903755,-0.499918702269186));
#131658=DIRECTION('',(0.978147600733807,-0.207911690817753,-1.3140998576179E-15));
#131659=DIRECTION('center_axis',(-0.207910764585316,-0.978147797608756,
-1.64014404456341E-6));
#131660=DIRECTION('ref_axis',(0.847118160920355,-0.180060523555695,0.49996902833652));
#131661=DIRECTION('',(0.489078856702179,-0.10395692016613,0.86602241926896));
#131662=DIRECTION('',(0.978147600733807,-0.207911690817753,-1.3140998576179E-15));
#131663=DIRECTION('center_axis',(0.207911690817753,0.978147600733807,6.85964567039975E-15));
#131664=DIRECTION('ref_axis',(2.78556626507032E-16,6.95368519647906E-15,
-1.));
#131665=DIRECTION('center_axis',(-0.207911690817752,-0.978147600733807,
2.89460408292303E-15));
#131666=DIRECTION('ref_axis',(0.855536389075788,-0.181849873245528,0.48475572257349));
#131667=DIRECTION('',(-0.518344070249267,0.110177433334231,-0.848045021223109));
#131668=DIRECTION('',(0.978147600733807,-0.207911690817753,-1.17328295072798E-15));
#131669=DIRECTION('',(-0.518344583061402,0.110177542335803,0.848044693619236));
#131670=DIRECTION('center_axis',(-0.207911690817764,-0.978147600733805,
-2.43973717020567E-14));
#131671=DIRECTION('ref_axis',(0.855538223422352,-0.181850263147927,-0.484752338886936));
#131672=DIRECTION('',(-0.978147600733807,0.207911690817753,1.3140998576179E-15));
#131673=DIRECTION('',(-0.489078856702203,0.103956920166127,-0.866022419268947));
#131674=DIRECTION('center_axis',(0.207912617177298,0.978147403828173,-1.64037041701691E-6));
#131675=DIRECTION('ref_axis',(0.84714667788718,-0.180066585252583,0.499918524381912));
#131676=DIRECTION('',(-0.978147600733807,0.207911690817753,1.3140998576179E-15));
#131677=DIRECTION('center_axis',(0.207910764792091,0.978147797564805,-1.63977752223453E-6));
#131678=DIRECTION('ref_axis',(0.847118057038102,-0.180060501475074,-0.499969212300654));
#131679=DIRECTION('',(-0.489078703542011,0.103956887610907,0.866022509672768));
#131680=DIRECTION('',(-0.978147600733807,0.207911690817753,1.3140998576179E-15));
#131681=DIRECTION('center_axis',(-2.80862404029962E-16,-6.96824330280696E-15,
1.));
#131682=DIRECTION('ref_axis',(-1.,1.96125168490647E-30,-2.80862404029962E-16));
#131683=DIRECTION('',(-0.994521895368274,0.104528463267647,4.49055953723918E-16));
#131684=DIRECTION('center_axis',(2.80862404029962E-16,6.96824330280696E-15,
-1.));
#131685=DIRECTION('ref_axis',(-1.,2.66453525910038E-15,-2.80862404029943E-16));
#131686=DIRECTION('',(0.994521895368274,-0.104528463267647,-4.49055953723918E-16));
#131687=DIRECTION('center_axis',(-2.80862404029962E-16,-6.96824330280696E-15,
1.));
#131688=DIRECTION('ref_axis',(-1.,2.09982394861192E-30,-2.80862404029962E-16));
#131689=DIRECTION('center_axis',(0.104528463267647,0.994521895368274,6.95942865237777E-15));
#131690=DIRECTION('ref_axis',(2.80862404029962E-16,6.96824330280696E-15,
-1.));
#131691=DIRECTION('center_axis',(0.104528463267647,0.994521895368274,3.92839035831992E-15));
#131692=DIRECTION('ref_axis',(0.869860024050247,-0.0914259726159766,-0.484752338922182));
#131693=DIRECTION('',(0.527021726387053,-0.0553922155202972,-0.848044693619247));
#131694=DIRECTION('',(-0.994521895368274,0.104528463267647,4.49055953723918E-16));
#131695=DIRECTION('',(0.527021204990422,-0.0553921607193138,0.8480450212231));
#131696=DIRECTION('center_axis',(0.104528463267653,0.994521895368273,1.72297862098881E-15));
#131697=DIRECTION('ref_axis',(0.869858159032045,-0.0914257765946727,0.484755722544297));
#131698=DIRECTION('',(0.994521895368274,-0.104528463267647,-5.89872860613828E-16));
#131699=DIRECTION('',(0.497265932938961,-0.0522647556052135,-0.866022509672741));
#131700=DIRECTION('center_axis',(-0.104529404915856,-0.994521796395256,
-1.63998887823304E-6));
#131701=DIRECTION('ref_axis',(0.861327901070945,-0.0905292105226773,-0.499918702269541));
#131702=DIRECTION('',(0.994521895368274,-0.104528463267647,-5.89872860613828E-16));
#131703=DIRECTION('center_axis',(-0.10452752153017,-0.994521994347068,-1.64014402515561E-6));
#131704=DIRECTION('ref_axis',(0.861299008823507,-0.0905261736006502,0.499969028333625));
#131705=DIRECTION('',(0.497266088663018,-0.0522647719724938,0.866022419268951));
#131706=DIRECTION('',(0.994521895368274,-0.104528463267647,-5.89872860613828E-16));
#131707=DIRECTION('center_axis',(0.104528463267647,0.994521895368274,6.95942865237777E-15));
#131708=DIRECTION('ref_axis',(2.80862404029962E-16,6.96824330280696E-15,
-1.));
#131709=DIRECTION('center_axis',(-0.104528463267644,-0.994521895368274,
-9.02840797292685E-15));
#131710=DIRECTION('ref_axis',(0.869858159015343,-0.0914257765929128,0.484755722574599));
#131711=DIRECTION('',(-0.527021204990403,0.0553921607193145,-0.848045021223112));
#131712=DIRECTION('',(0.994521895368274,-0.104528463267647,-4.49055953723918E-16));
#131713=DIRECTION('',(-0.527021726387063,0.0553922155202998,0.848044693619241));
#131714=DIRECTION('center_axis',(-0.104528463267641,-0.994521895368275,
3.7216329714999E-15));
#131715=DIRECTION('ref_axis',(0.869860024068749,-0.0914259726179193,-0.484752338888615));
#131716=DIRECTION('',(-0.994521895368274,0.104528463267647,5.89872860613828E-16));
#131717=DIRECTION('',(-0.49726608866303,0.0522647719724906,-0.866022419268944));
#131718=DIRECTION('center_axis',(0.104529405134737,0.99452179637225,-1.6403704179208E-6));
#131719=DIRECTION('ref_axis',(0.861328003191142,-0.090529221256205,0.499918524379227));
#131720=DIRECTION('',(-0.994521895368274,0.104528463267647,5.89872860613828E-16));
#131721=DIRECTION('center_axis',(0.104527521740381,0.994521994324975,-1.6397775587696E-6));
#131722=DIRECTION('ref_axis',(0.861298903200557,-0.0905261624994676,-0.499969212300755));
#131723=DIRECTION('',(-0.497265932938963,0.0522647556052233,0.866022509672739));
#131724=DIRECTION('',(-0.994521895368274,0.104528463267647,5.89872860613828E-16));
#131725=DIRECTION('center_axis',(-2.81633813779821E-16,-6.98296267768627E-15,
1.));
#131726=DIRECTION('ref_axis',(-1.,1.96663841039893E-30,-2.81633813779821E-16));
#131727=DIRECTION('',(-1.,1.96663841039893E-30,-2.81633813779821E-16));
#131728=DIRECTION('',(1.,-1.96663841039893E-30,2.81633813779821E-16));
#131729=DIRECTION('center_axis',(0.,1.,6.98296267768627E-15));
#131730=DIRECTION('ref_axis',(2.81633813779821E-16,6.98296267768627E-15,
-1.));
#131731=DIRECTION('center_axis',(2.50576143790467E-16,1.,7.42579081592464E-15));
#131732=DIRECTION('ref_axis',(0.874651456242924,3.38050267731257E-15,-0.48475233892384));
#131733=DIRECTION('',(0.529924709392056,5.93414301348777E-15,-0.848044693619236));
#131734=DIRECTION('',(-1.,1.96663841039893E-30,-2.81633813779821E-16));
#131735=DIRECTION('',(0.529924185123406,-5.93414530587669E-15,0.848045021223104));
#131736=DIRECTION('center_axis',(-2.50577545723561E-16,1.,7.42579288222807E-15));
#131737=DIRECTION('ref_axis',(0.874649580953153,-3.38052804871796E-15,0.484755722543297));
#131738=DIRECTION('',(1.,-9.83319205199467E-31,1.40816906889911E-16));
#131739=DIRECTION('',(0.500005012714991,5.91835148258668E-15,-0.866022509672746));
#131740=DIRECTION('center_axis',(-9.46835262596884E-7,-0.999999999998207,
-1.63998887409855E-6));
#131741=DIRECTION('ref_axis',(0.866072335963508,-1.66717974320025E-10,-0.499918702269391));
#131742=DIRECTION('',(1.,-9.83319205199467E-31,1.40816906889911E-16));
#131743=DIRECTION('center_axis',(9.46924640381337E-7,-0.999999999998207,
-1.64014403445674E-6));
#131744=DIRECTION('ref_axis',(0.866043284544476,5.65065332453387E-11,0.499969028336172));
#131745=DIRECTION('',(0.50000516929686,-5.91835086477054E-15,0.866022419268935));
#131746=DIRECTION('',(1.,-9.83319205199467E-31,1.40816906889911E-16));
#131747=DIRECTION('center_axis',(0.,1.,6.98296267768627E-15));
#131748=DIRECTION('ref_axis',(2.81633813779821E-16,6.98296267768627E-15,
-1.));
#131749=DIRECTION('center_axis',(5.53239297233671E-17,-1.,-7.21882753498418E-15));
#131750=DIRECTION('ref_axis',(0.874649580936035,-3.45097890591139E-15,0.484755722574184));
#131751=DIRECTION('',(-0.529924185123415,5.88254404234729E-15,-0.848045021223098));
#131752=DIRECTION('',(1.,-1.96663841039893E-30,2.81633813779821E-16));
#131753=DIRECTION('',(-0.529924709392047,-5.88254176989226E-15,0.848044693619242));
#131754=DIRECTION('center_axis',(-5.53227018708228E-17,-1.,-7.21882542204734E-15));
#131755=DIRECTION('ref_axis',(0.874651456262773,3.45095442560608E-15,-0.484752338888025));
#131756=DIRECTION('',(-1.,9.83319205199467E-31,-1.40816906889911E-16));
#131757=DIRECTION('',(-0.50000516929686,6.05598693139311E-15,-0.866022419268935));
#131758=DIRECTION('center_axis',(9.47055349398689E-7,0.999999999998206,
-1.64037041837183E-6));
#131759=DIRECTION('ref_axis',(0.866072438647096,-1.66977002397838E-10,0.499918524377595));
#131760=DIRECTION('',(-1.,9.83319205199467E-31,-1.40816906889911E-16));
#131761=DIRECTION('center_axis',(-9.46713274170111E-7,0.999999999998207,
-1.63977756707643E-6));
#131762=DIRECTION('ref_axis',(0.866043178342101,5.62743837908293E-11,-0.499969212299229));
#131763=DIRECTION('',(-0.500005012714993,-6.05598756357666E-15,0.866022509672745));
#131764=DIRECTION('',(-1.,9.83319205199467E-31,-1.40816906889911E-16));
#131765=DIRECTION('center_axis',(-2.80862404029962E-16,-6.99768205256557E-15,
1.));
#131766=DIRECTION('ref_axis',(-1.,1.96125168490646E-30,-2.80862404029962E-16));
#131767=DIRECTION('',(-0.994521895368273,-0.104528463267661,-1.01078076178394E-15));
#131768=DIRECTION('center_axis',(2.80862404029962E-16,6.99768205256557E-15,
-1.));
#131769=DIRECTION('ref_axis',(-1.,-2.29860575018392E-12,-2.80862404046047E-16));
#131770=DIRECTION('',(0.994521895368273,0.104528463267661,1.01078076178394E-15));
#131771=DIRECTION('center_axis',(-2.80862404029962E-16,-6.99768205256557E-15,
1.));
#131772=DIRECTION('ref_axis',(-1.,2.09987333638716E-30,-2.80862404029962E-16));
#131773=DIRECTION('center_axis',(-0.104528463267661,0.994521895368273,6.92998990261915E-15));
#131774=DIRECTION('ref_axis',(2.80862404029962E-16,6.99768205256558E-15,
-1.));
#131775=DIRECTION('center_axis',(-0.104528463267665,0.994521895368272,-3.99730948741319E-15));
#131776=DIRECTION('ref_axis',(0.869860024049594,0.0914259726159237,-0.484752338923364));
#131777=DIRECTION('',(0.527021726387062,0.0553922155203198,-0.84804469361924));
#131778=DIRECTION('',(-0.994521895368273,-0.104528463267661,-1.01078076178394E-15));
#131779=DIRECTION('',(0.527021204990404,0.0553921607193099,0.848045021223112));
#131780=DIRECTION('center_axis',(-0.104528463267673,0.994521895368271,2.43973772732041E-14));
#131781=DIRECTION('ref_axis',(0.869858159031862,0.0914257765946581,0.484755722544626));
#131782=DIRECTION('',(0.994521895368273,0.104528463267661,8.69963854894025E-16));
#131783=DIRECTION('',(0.497265932938987,0.0522647556052302,-0.866022509672725));
#131784=DIRECTION('center_axis',(0.104527521619062,-0.994521994337725,-1.63998890568842E-6));
#131785=DIRECTION('ref_axis',(0.861327901104011,0.0905292101909037,-0.499918702272649));
#131786=DIRECTION('',(0.994521895368273,0.104528463267661,8.69963854894025E-16));
#131787=DIRECTION('center_axis',(0.104529405004759,-0.994521796385912,-1.6401440355691E-6));
#131788=DIRECTION('ref_axis',(0.861299008813094,0.0905261737132066,0.499969028331184));
#131789=DIRECTION('',(0.497266088663019,0.0522647719724762,0.866022419268952));
#131790=DIRECTION('',(0.994521895368273,0.104528463267661,8.69963854894025E-16));
#131791=DIRECTION('center_axis',(-0.104528463267661,0.994521895368273,6.92998990261915E-15));
#131792=DIRECTION('ref_axis',(2.80862404029962E-16,6.99768205256558E-15,
-1.));
#131793=DIRECTION('center_axis',(0.104528463267666,-0.994521895368272,-2.20541263460803E-14));
#131794=DIRECTION('ref_axis',(0.86985815901466,0.0914257765928456,0.484755722575836));
#131795=DIRECTION('',(-0.527021204990422,-0.0553921607193138,-0.8480450212231));
#131796=DIRECTION('',(0.994521895368273,0.104528463267661,1.01078076178394E-15));
#131797=DIRECTION('',(-0.527021726387058,-0.0553922155203158,0.848044693619243));
#131798=DIRECTION('center_axis',(0.10452846326766,-0.994521895368273,-7.96015941126447E-15));
#131799=DIRECTION('ref_axis',(0.869860024068839,0.0914259726179483,-0.484752338888448));
#131800=DIRECTION('',(-0.994521895368273,-0.104528463267661,-8.69963854894025E-16));
#131801=DIRECTION('',(-0.497266088663004,-0.0522647719724695,-0.866022419268961));
#131802=DIRECTION('center_axis',(-0.104527521400179,0.99452199436073,-1.64037044554758E-6));
#131803=DIRECTION('ref_axis',(0.861328003227402,0.0905292209242402,0.499918524376869));
#131804=DIRECTION('',(-0.994521895368273,-0.104528463267661,-8.69963854894025E-16));
#131805=DIRECTION('center_axis',(-0.104529404794561,0.994521796408005,-1.63977758411593E-6));
#131806=DIRECTION('ref_axis',(0.861298903191925,0.0905261626117421,-0.499969212295296));
#131807=DIRECTION('',(-0.497265932938963,-0.0522647556052321,0.866022509672738));
#131808=DIRECTION('',(-0.994521895368273,-0.104528463267661,-8.69963854894025E-16));
#131809=DIRECTION('center_axis',(-2.78556626507032E-16,-7.01224015889348E-15,
1.));
#131810=DIRECTION('ref_axis',(-1.,1.9451505265208E-30,-2.78556626507032E-16));
#131811=DIRECTION('',(-0.978147600733804,-0.207911690817766,-1.73039620374214E-15));
#131812=DIRECTION('center_axis',(2.78556626507032E-16,7.01224015889348E-15,
-1.));
#131813=DIRECTION('ref_axis',(-1.,-2.43272069155864E-12,-2.78556626524091E-16));
#131814=DIRECTION('',(0.978147600733804,0.207911690817766,1.73039620374214E-15));
#131815=DIRECTION('center_axis',(-2.78556626507032E-16,-7.01224015889348E-15,
1.));
#131816=DIRECTION('ref_axis',(-1.,2.08372909397962E-30,-2.78556626507032E-16));
#131817=DIRECTION('center_axis',(-0.207911690817766,0.978147600733804,6.80109070798531E-15));
#131818=DIRECTION('ref_axis',(2.78556626507032E-16,7.01224015889348E-15,
-1.));
#131819=DIRECTION('center_axis',(-0.207911690817786,0.9781476007338,-2.72919751209605E-14));
#131820=DIRECTION('ref_axis',(0.855538223402316,0.181850263143686,-0.48475233892389));
#131821=DIRECTION('',(0.518344583061382,0.110177542335822,-0.848044693619246));
#131822=DIRECTION('',(-0.978147600733804,-0.207911690817766,-1.73039620374214E-15));
#131823=DIRECTION('',(0.518344070249262,0.110177433334227,0.848045021223113));
#131824=DIRECTION('center_axis',(-0.207911690817754,0.978147600733807,-2.06757434518659E-14));
#131825=DIRECTION('ref_axis',(0.855536389092255,0.181849873249041,0.484755722543111));
#131826=DIRECTION('',(0.978147600733804,0.207911690817766,1.58957929685223E-15));
#131827=DIRECTION('',(0.489078703542061,0.103956887610937,-0.866022509672736));
#131828=DIRECTION('center_axis',(0.207910764672762,-0.978147797590169,-1.63998887332749E-6));
#131829=DIRECTION('ref_axis',(0.847146577520758,0.18006656357791,-0.499918702266787));
#131830=DIRECTION('',(0.978147600733804,0.207911690817766,1.58957929685223E-15));
#131831=DIRECTION('center_axis',(0.207912617049462,-0.978147403855346,-1.64014402838238E-6));
#131832=DIRECTION('ref_axis',(0.847118160900355,0.180060523666994,0.499969028330324));
#131833=DIRECTION('',(0.489078856702179,0.10395692016613,0.86602241926896));
#131834=DIRECTION('',(0.978147600733804,0.207911690817766,1.58957929685223E-15));
#131835=DIRECTION('center_axis',(-0.207911690817766,0.978147600733804,6.80109070798531E-15));
#131836=DIRECTION('ref_axis',(2.78556626507032E-16,7.01224015889348E-15,
-1.));
#131837=DIRECTION('center_axis',(0.207911690817764,-0.978147600733805,-1.32324758076486E-14));
#131838=DIRECTION('ref_axis',(0.855536389075988,0.181849873245576,0.48475572257312));
#131839=DIRECTION('',(-0.518344070249253,-0.110177433334228,-0.848045021223118));
#131840=DIRECTION('',(0.978147600733804,0.207911690817766,1.73039620374214E-15));
#131841=DIRECTION('',(-0.518344583061406,-0.11017754233582,0.848044693619231));
#131842=DIRECTION('center_axis',(0.207911690817771,-0.978147600733803,-1.60581570807317E-14));
#131843=DIRECTION('ref_axis',(0.855538223422078,0.181850263147895,-0.484752338887433));
#131844=DIRECTION('',(-0.978147600733804,-0.207911690817766,-1.58957929685223E-15));
#131845=DIRECTION('',(-0.489078856702194,-0.103956920166107,-0.866022419268955));
#131846=DIRECTION('center_axis',(-0.20791076445747,0.97814779763593,-1.64037044223425E-6));
#131847=DIRECTION('ref_axis',(0.847146677959787,0.18006658492662,0.499918524376283));
#131848=DIRECTION('',(-0.978147600733804,-0.207911690817766,-1.58957929685223E-15));
#131849=DIRECTION('center_axis',(-0.207912616842705,0.978147403899295,-1.63977754289028E-6));
#131850=DIRECTION('ref_axis',(0.847118057015926,0.180060501585439,-0.49996921229848));
#131851=DIRECTION('',(-0.489078703542037,-0.103956887610949,0.866022509672748));
#131852=DIRECTION('',(-0.978147600733804,-0.207911690817766,-1.58957929685223E-15));
#131853=DIRECTION('center_axis',(-2.74741743792087E-16,-7.02647749501056E-15,
1.));
#131854=DIRECTION('ref_axis',(-1.,1.91851134290259E-30,-2.74741743792087E-16));
#131855=DIRECTION('',(-0.951056516295151,-0.309016994374954,-2.43259588228318E-15));
#131856=DIRECTION('center_axis',(2.74741743792087E-16,7.02647749501057E-15,
-1.));
#131857=DIRECTION('ref_axis',(-1.,-2.73292499741728E-12,-2.7474174381129E-16));
#131858=DIRECTION('',(0.951056516295151,0.309016994374954,2.43259588228318E-15));
#131859=DIRECTION('center_axis',(-2.74741743792087E-16,-7.02647749501057E-15,
1.));
#131860=DIRECTION('ref_axis',(-1.,2.1085382641719E-30,-2.74741743792087E-16));
#131861=DIRECTION('center_axis',(-0.309016994374955,0.951056516295151,6.59767734033506E-15));
#131862=DIRECTION('ref_axis',(2.74741743792088E-16,7.02647749501057E-15,
-1.));
#131863=DIRECTION('center_axis',(-0.309016994374942,0.951056516295155,3.83190357758892E-14));
#131864=DIRECTION('ref_axis',(0.831842966947115,0.270282164133951,-0.484752338923381));
#131865=DIRECTION('',(0.503988348013127,0.16375574094136,-0.848044693619237));
#131866=DIRECTION('',(-0.951056516295151,-0.309016994374955,-2.43259588228318E-15));
#131867=DIRECTION('',(0.503987849404007,0.163755578933431,0.848045021223107));
#131868=DIRECTION('center_axis',(-0.309016994374941,0.951056516295156,-1.19919312020825E-14));
#131869=DIRECTION('ref_axis',(0.831841183439686,0.270281584637244,0.484755722544503));
#131870=DIRECTION('',(0.951056516295151,0.309016994374955,2.29177897539327E-15));
#131871=DIRECTION('',(0.47553302552288,0.15451004620161,-0.866022509672718));
#131872=DIRECTION('center_axis',(0.309016093880556,-0.951056808881632,-1.63998887048721E-6));
#131873=DIRECTION('ref_axis',(0.823683738754044,0.267631070012658,-0.499918702266717));
#131874=DIRECTION('',(0.951056516295151,0.309016994374955,2.29177897539327E-15));
#131875=DIRECTION('center_axis',(0.309017894953215,-0.951056223677651,-1.64014397020222E-6));
#131876=DIRECTION('ref_axis',(0.823656109144283,0.267622092842959,0.499969028332411));
#131877=DIRECTION('',(0.475533174441003,0.154510094588037,0.866022419268958));
#131878=DIRECTION('',(0.951056516295151,0.309016994374955,2.29177897539327E-15));
#131879=DIRECTION('center_axis',(-0.309016994374955,0.951056516295151,6.59767734033506E-15));
#131880=DIRECTION('ref_axis',(2.74741743792088E-16,7.02647749501057E-15,
-1.));
#131881=DIRECTION('center_axis',(0.309016994374966,-0.951056516295147,-4.13514868989001E-14));
#131882=DIRECTION('ref_axis',(0.831841183424408,0.270281584632277,0.484755722573489));
#131883=DIRECTION('',(-0.503987849403998,-0.163755578933433,-0.848045021223113));
#131884=DIRECTION('',(0.951056516295151,0.309016994374955,2.43259588228318E-15));
#131885=DIRECTION('',(-0.503988348013108,-0.163755740941352,0.84804469361925));
#131886=DIRECTION('center_axis',(0.30901699437492,-0.951056516295162,-7.37434681389843E-14));
#131887=DIRECTION('ref_axis',(0.831842966966455,0.270282164140231,-0.484752338886692));
#131888=DIRECTION('',(-0.951056516295151,-0.309016994374955,-2.29177897539327E-15));
#131889=DIRECTION('',(-0.475533174441042,-0.154510094588038,-0.866022419268936));
#131890=DIRECTION('center_axis',(-0.309016093671208,0.951056808949653,-1.6403705334645E-6));
#131891=DIRECTION('ref_axis',(0.823683836411346,0.267631101743197,0.499918524376132));
#131892=DIRECTION('',(-0.951056516295151,-0.309016994374955,-2.29177897539327E-15));
#131893=DIRECTION('center_axis',(-0.309017894752207,0.951056223742963,-1.63977755898441E-6));
#131894=DIRECTION('ref_axis',(0.823656008137761,0.26762206002369,-0.499969212299362));
#131895=DIRECTION('',(-0.475533025522815,-0.154510046201603,0.866022509672754));
#131896=DIRECTION('',(-0.951056516295151,-0.309016994374955,-2.29177897539327E-15));
#131897=DIRECTION('center_axis',(-2.69459552538469E-16,-7.04023807368299E-15,
1.));
#131898=DIRECTION('ref_axis',(-1.,1.88162599852217E-30,-2.69459552538469E-16));
#131899=DIRECTION('',(-0.913545457642598,-0.406736643075807,-3.10968635078423E-15));
#131900=DIRECTION('center_axis',(2.69459552538469E-16,7.04023807368299E-15,
-1.));
#131901=DIRECTION('ref_axis',(-1.,-1.34203759216689E-12,-2.69459552547917E-16));
#131902=DIRECTION('',(0.913545457642598,0.406736643075807,3.10968635078423E-15));
#131903=DIRECTION('center_axis',(-2.69459552538469E-16,-7.04023807368299E-15,
1.));
#131904=DIRECTION('ref_axis',(-1.,2.07139034025888E-30,-2.69459552538469E-16));
#131905=DIRECTION('center_axis',(-0.406736643075807,0.913545457642598,6.32197843909136E-15));
#131906=DIRECTION('ref_axis',(2.69459552538469E-16,7.04023807368299E-15,
-1.));
#131907=DIRECTION('center_axis',(-0.406736643075815,0.913545457642594,9.64867807306692E-15));
#131908=DIRECTION('ref_axis',(0.799033864871477,0.355752797173747,-0.484752338923296));
#131909=DIRECTION('',(0.484110311157675,0.215539797381046,-0.848044693619243));
#131910=DIRECTION('',(-0.913545457642598,-0.406736643075807,-3.10968635078423E-15));
#131911=DIRECTION('',(0.484109832214418,0.215539584141762,0.848045021223121));
#131912=DIRECTION('center_axis',(-0.406736643075818,0.913545457642593,2.68784664874263E-14));
#131913=DIRECTION('ref_axis',(0.799032151707959,0.35575203442419,0.484755722544869));
#131914=DIRECTION('',(0.913545457642598,0.406736643075807,2.96886944389432E-15));
#131915=DIRECTION('',(0.456777308164318,0.203370360392767,-0.866022509672743));
#131916=DIRECTION('center_axis',(0.406735778098062,-0.913545842753539,-1.63998876755266E-6));
#131917=DIRECTION('ref_axis',(0.791196448576301,0.352263354437902,-0.499918702271085));
#131918=DIRECTION('',(0.913545457642598,0.406736643075807,2.96886944389432E-15));
#131919=DIRECTION('center_axis',(0.406737508133866,-0.913545072491972,-1.64014417590034E-6));
#131920=DIRECTION('ref_axis',(0.791169908699022,0.352251538367612,0.499969028327587));
#131921=DIRECTION('',(0.456777451208935,0.203370424080325,0.866022419268958));
#131922=DIRECTION('',(0.913545457642598,0.406736643075807,2.96886944389432E-15));
#131923=DIRECTION('center_axis',(-0.406736643075807,0.913545457642598,6.32197843909136E-15));
#131924=DIRECTION('ref_axis',(2.69459552538469E-16,7.04023807368299E-15,
-1.));
#131925=DIRECTION('center_axis',(0.406736643075821,-0.913545457642592,-5.01731374373328E-14));
#131926=DIRECTION('ref_axis',(0.799032151694043,0.355752034417985,0.484755722572362));
#131927=DIRECTION('',(-0.484109832214425,-0.215539584141772,-0.848045021223115));
#131928=DIRECTION('',(0.913545457642598,0.406736643075807,3.10968635078423E-15));
#131929=DIRECTION('',(-0.484110311157673,-0.215539797381045,0.848044693619245));
#131930=DIRECTION('center_axis',(0.406736643075753,-0.913545457642622,-9.74516485500229E-14));
#131931=DIRECTION('ref_axis',(0.799033864889399,0.355752797181708,-0.484752338887911));
#131932=DIRECTION('',(-0.913545457642598,-0.406736643075807,-2.96886944389432E-15));
#131933=DIRECTION('',(-0.456777451208932,-0.203370424080342,-0.866022419268955));
#131934=DIRECTION('center_axis',(-0.406735777896963,0.913545842843073,-1.64037041701662E-6));
#131935=DIRECTION('ref_axis',(0.791196542384111,0.352263396203563,0.499918524376282));
#131936=DIRECTION('',(-0.913545457642598,-0.406736643075807,-2.96886944389432E-15));
#131937=DIRECTION('center_axis',(-0.406737507940739,0.913545072577959,-1.63977763214104E-6));
#131938=DIRECTION('ref_axis',(0.791169811676832,0.352251495170301,-0.499969212293651));
#131939=DIRECTION('',(-0.456777308164302,-0.203370360392813,0.86602250967274));
#131940=DIRECTION('',(-0.913545457642598,-0.406736643075807,-2.96886944389432E-15));
#131941=DIRECTION('center_axis',(-2.6276792553892E-16,-7.05337113113122E-15,
1.));
#131942=DIRECTION('ref_axis',(-1.,1.83489861693132E-30,-2.6276792553892E-16));
#131943=DIRECTION('',(-0.866025403784435,-0.500000000000007,-3.7542492643821E-15));
#131944=DIRECTION('center_axis',(2.6276792553892E-16,7.05337113113122E-15,
-1.));
#131945=DIRECTION('ref_axis',(-1.,1.96511414759077E-30,-2.6276792553892E-16));
#131946=DIRECTION('',(0.866025403784435,0.500000000000007,3.7542492643821E-15));
#131947=DIRECTION('center_axis',(-2.6276792553892E-16,-7.05337113113122E-15,
1.));
#131948=DIRECTION('ref_axis',(-1.,1.6583547235129E-30,-2.6276792553892E-16));
#131949=DIRECTION('center_axis',(-0.500000000000007,0.866025403784435,5.97701461910993E-15));
#131950=DIRECTION('ref_axis',(2.6276792553892E-16,7.05337113113122E-15,
-1.));
#131951=DIRECTION('center_axis',(-0.500000000000001,0.866025403784438,3.85947122922661E-15));
#131952=DIRECTION('ref_axis',(0.757470380563486,0.4373257281215,-0.484752338923709));
#131953=DIRECTION('',(0.458928260426603,0.264962354696026,-0.848044693619239));
#131954=DIRECTION('',(-0.866025403784435,-0.500000000000007,-3.7542492643821E-15));
#131955=DIRECTION('',(0.458927806396619,0.264962092561704,0.848045021223113));
#131956=DIRECTION('center_axis',(-0.49999999999998,0.86602540378445,-3.36325426817014E-14));
#131957=DIRECTION('ref_axis',(0.757468756514423,0.437324790476329,0.484755722544178));
#131958=DIRECTION('',(0.866025403784435,0.500000000000007,3.61343235749219E-15));
#131959=DIRECTION('',(0.433017043030755,0.250002506357519,-0.866022509672733));
#131960=DIRECTION('center_axis',(0.499999180015738,-0.866025877200503,-1.63998885396272E-6));
#131961=DIRECTION('ref_axis',(0.750040644542557,0.433036167837314,-0.499918702269639));
#131962=DIRECTION('',(0.866025403784435,0.500000000000007,3.61343235749219E-15));
#131963=DIRECTION('center_axis',(0.500000820059927,-0.866024930320548,-1.64014403113693E-6));
#131964=DIRECTION('ref_axis',(0.75001548516595,0.433021642322233,0.499969028332597));
#131965=DIRECTION('',(0.433017178634557,0.250002584648415,0.86602241926897));
#131966=DIRECTION('',(0.866025403784435,0.500000000000007,3.61343235749219E-15));
#131967=DIRECTION('center_axis',(-0.500000000000007,0.866025403784435,5.97701461910993E-15));
#131968=DIRECTION('ref_axis',(2.6276792553892E-16,7.05337113113122E-15,
-1.));
#131969=DIRECTION('center_axis',(0.499999999999989,-0.866025403784445,4.74163716440701E-14));
#131970=DIRECTION('ref_axis',(0.757468756500261,0.437324790468171,0.484755722573669));
#131971=DIRECTION('',(-0.458927806396633,-0.264962092561691,-0.848045021223109));
#131972=DIRECTION('',(0.866025403784435,0.500000000000007,3.7542492643821E-15));
#131973=DIRECTION('',(-0.458928260426587,-0.264962354696025,0.848044693619248));
#131974=DIRECTION('center_axis',(0.499999999999975,-0.866025403784453,-5.47217885068692E-14));
#131975=DIRECTION('ref_axis',(0.757470380580527,0.437325728131337,-0.484752338888207));
#131976=DIRECTION('',(-0.866025403784435,-0.500000000000007,-3.61343235749219E-15));
#131977=DIRECTION('',(-0.433017178634597,-0.250002584648401,-0.866022419268954));
#131978=DIRECTION('center_axis',(-0.499999179825182,0.866025877310519,-1.64037034334471E-6));
#131979=DIRECTION('ref_axis',(0.75004073347165,0.433036219180271,0.499918524373088));
#131980=DIRECTION('',(-0.866025403784435,-0.500000000000007,-3.61343235749219E-15));
#131981=DIRECTION('center_axis',(-0.500000819876911,0.866024930426213,-1.63977768085434E-6));
#131982=DIRECTION('ref_axis',(0.750015393190062,0.433021589219632,-0.499969212299778));
#131983=DIRECTION('',(-0.433017043030724,-0.250002506357501,0.866022509672754));
#131984=DIRECTION('',(-0.866025403784435,-0.500000000000007,-3.61343235749219E-15));
#131985=DIRECTION('center_axis',(-2.54740177659162E-16,-7.0657327788296E-15,
1.));
#131986=DIRECTION('ref_axis',(-1.,1.7788411531011E-30,-2.54740177659162E-16));
#131987=DIRECTION('',(-0.809016994374943,-0.58778525229248,-4.35922265691196E-15));
#131988=DIRECTION('center_axis',(2.54740177659162E-16,7.0657327788296E-15,
-1.));
#131989=DIRECTION('ref_axis',(-1.,-1.29496413592278E-12,-2.54740177668312E-16));
#131990=DIRECTION('',(0.809016994374943,0.58778525229248,4.35922265691196E-15));
#131991=DIRECTION('center_axis',(-2.54740177659162E-16,-7.0657327788296E-15,
1.));
#131992=DIRECTION('ref_axis',(-1.,1.65352321226724E-30,-2.54740177659162E-16));
#131993=DIRECTION('center_axis',(-0.58778525229248,0.809016994374943,5.56656537619081E-15));
#131994=DIRECTION('ref_axis',(2.54740177659162E-16,7.0657327788296E-15,
-1.));
#131995=DIRECTION('center_axis',(-0.587785252292507,0.809016994374923,-8.68381026576039E-14));
#131996=DIRECTION('ref_axis',(0.707607892255758,0.514107226876036,-0.484752338922871));
#131997=DIRECTION('',(0.42871809563737,0.311481929006034,-0.848044693619238));
#131998=DIRECTION('',(-0.809016994374943,-0.58778525229248,-4.35922265691196E-15));
#131999=DIRECTION('',(0.42871767149512,0.31148162084863,0.848045021223115));
#132000=DIRECTION('center_axis',(-0.58778525229246,0.809016994374957,-2.37081858248059E-14));
#132001=DIRECTION('ref_axis',(0.707606375114078,0.514106124608088,0.484755722543188));
#132002=DIRECTION('',(0.809016994374943,0.58778525229248,4.21840575002205E-15));
#132003=DIRECTION('',(0.404512552559089,0.293895572546202,-0.86602250967274));
#132004=DIRECTION('center_axis',(0.587784486285637,-0.809017550909275,-1.63998885809377E-6));
#132005=DIRECTION('ref_axis',(0.700667238250818,0.509064546363247,-0.499918702268632));
#132006=DIRECTION('',(0.809016994374943,0.58778525229248,4.21840575002205E-15));
#132007=DIRECTION('center_axis',(0.587786018369622,-0.809016437785102,-1.64014417882589E-6));
#132008=DIRECTION('ref_axis',(0.700643735030366,0.509047470549938,0.499969028330164));
#132009=DIRECTION('',(0.404512679236484,0.293895664582674,0.866022419268941));
#132010=DIRECTION('',(0.809016994374943,0.58778525229248,4.21840575002205E-15));
#132011=DIRECTION('center_axis',(-0.58778525229248,0.809016994374943,5.56656537619081E-15));
#132012=DIRECTION('ref_axis',(2.54740177659162E-16,7.0657327788296E-15,
-1.));
#132013=DIRECTION('center_axis',(0.587785252292496,-0.809016994374931,3.85947211056421E-15));
#132014=DIRECTION('ref_axis',(0.707606375100321,0.514106124598129,0.484755722573831));
#132015=DIRECTION('',(-0.428717671495122,-0.311481620848618,-0.848045021223118));
#132016=DIRECTION('',(0.809016994374943,0.58778525229248,4.35922265691196E-15));
#132017=DIRECTION('',(-0.428718095637371,-0.311481929006031,0.848044693619239));
#132018=DIRECTION('center_axis',(0.587785252292485,-0.809016994374939,-2.16406065379816E-14));
#132019=DIRECTION('ref_axis',(0.707607892271911,0.514107226887808,-0.484752338886809));
#132020=DIRECTION('',(-0.809016994374942,-0.58778525229248,-4.21840575002204E-15));
#132021=DIRECTION('',(-0.404512679236477,-0.293895664582651,-0.866022419268952));
#132022=DIRECTION('center_axis',(-0.587784486107578,0.809017551038641,-1.64037040754943E-6));
#132023=DIRECTION('ref_axis',(0.7006673213238,0.509064606718979,0.499918524376705));
#132024=DIRECTION('',(-0.809016994374943,-0.58778525229248,-4.21840575002205E-15));
#132025=DIRECTION('center_axis',(-0.587786018198513,0.809016437909421,-1.63977749787816E-6));
#132026=DIRECTION('ref_axis',(0.700643649108078,0.50904740812344,-0.499969212299442));
#132027=DIRECTION('',(-0.404512552559112,-0.293895572546185,0.866022509672735));
#132028=DIRECTION('',(-0.809016994374943,-0.58778525229248,-4.21840575002205E-15));
#132029=DIRECTION('center_axis',(-2.45464262584879E-16,-7.07718757997909E-15,
1.));
#132030=DIRECTION('ref_axis',(-1.,1.71406778433599E-30,-2.45464262584879E-16));
#132031=DIRECTION('',(-0.743144825477389,-0.669130606358864,-4.91797831328641E-15));
#132032=DIRECTION('center_axis',(2.45464262584879E-16,7.07718757997909E-15,
-1.));
#132033=DIRECTION('ref_axis',(-1.,7.62234719786647E-12,-2.45464262530934E-16));
#132034=DIRECTION('',(0.743144825477389,0.669130606358864,4.91797831328641E-15));
#132035=DIRECTION('center_axis',(-2.45464262584879E-16,-7.07718757997909E-15,
1.));
#132036=DIRECTION('ref_axis',(-1.,1.691840019653E-30,-2.45464262584879E-16));
#132037=DIRECTION('center_axis',(-0.669130606358865,0.743144825477389,5.09512767813145E-15));
#132038=DIRECTION('ref_axis',(2.45464262584878E-16,7.07718757997909E-15,
-1.));
#132039=DIRECTION('center_axis',(-0.66913060635884,0.743144825477411,4.41082426197315E-14));
#132040=DIRECTION('ref_axis',(0.649992703804842,0.585256059269967,-0.484752338919845));
#132041=DIRECTION('',(0.393810805677312,0.35458884212006,-0.848044693619234));
#132042=DIRECTION('',(-0.743144825477389,-0.669130606358864,-4.91797831328641E-15));
#132043=DIRECTION('',(0.393810416069775,0.354588491315832,0.848045021223115));
#132044=DIRECTION('center_axis',(-0.669130606358884,0.743144825477371,3.99731040069399E-14));
#132045=DIRECTION('ref_axis',(0.649991310190922,0.585254804454373,0.484755722544212));
#132046=DIRECTION('',(0.743144825477389,0.669130606358864,4.7771614063965E-15));
#132047=DIRECTION('',(0.371576137911922,0.334568657340493,-0.866022509672722));
#132048=DIRECTION('center_axis',(0.669129902721978,-0.743145459032475,-1.63998882521664E-6));
#132049=DIRECTION('ref_axis',(0.643617175072631,0.579515507190644,-0.499918702267776));
#132050=DIRECTION('',(0.743144825477389,0.669130606358864,4.7771614063965E-15));
#132051=DIRECTION('center_axis',(0.669131310059903,-0.743144191859714,-1.64014420739982E-6));
#132052=DIRECTION('ref_axis',(0.643595585511274,0.579496068162662,0.499969028335171));
#132053=DIRECTION('',(0.371576254274849,0.334568762114141,0.866022419268973));
#132054=DIRECTION('',(0.743144825477389,0.669130606358864,4.7771614063965E-15));
#132055=DIRECTION('center_axis',(-0.669130606358865,0.743144825477389,5.09512767813145E-15));
#132056=DIRECTION('ref_axis',(2.45464262584878E-16,7.07718757997909E-15,
-1.));
#132057=DIRECTION('center_axis',(0.669130606358884,-0.743144825477371,-6.75407619348748E-14));
#132058=DIRECTION('ref_axis',(0.649991310179477,0.58525480444405,0.484755722572022));
#132059=DIRECTION('',(-0.393810416069763,-0.354588491315834,-0.848045021223119));
#132060=DIRECTION('',(0.743144825477389,0.669130606358864,4.91797831328641E-15));
#132061=DIRECTION('',(-0.39381080567731,-0.354588842120051,0.848044693619239));
#132062=DIRECTION('center_axis',(0.669130606358841,-0.74314482547741,-5.76163919291452E-14));
#132063=DIRECTION('ref_axis',(0.64999270381715,0.585256059281061,-0.484752338889947));
#132064=DIRECTION('',(-0.743144825477389,-0.669130606358864,-4.7771614063965E-15));
#132065=DIRECTION('',(-0.371576254274891,-0.334568762114186,-0.866022419268937));
#132066=DIRECTION('center_axis',(-0.669129902558376,0.743145459179781,-1.64037043577932E-6));
#132067=DIRECTION('ref_axis',(0.643617251383537,0.579515575900918,0.49991852437145));
#132068=DIRECTION('',(-0.743144825477389,-0.669130606358864,-4.7771614063965E-15));
#132069=DIRECTION('center_axis',(-0.669131309902728,0.743144192001237,-1.63977757912426E-6));
#132070=DIRECTION('ref_axis',(0.643595506588524,0.579495997099938,-0.499969212296327));
#132071=DIRECTION('',(-0.371576137911874,-0.334568657340446,0.866022509672761));
#132072=DIRECTION('',(-0.743144825477389,-0.669130606358864,-4.7771614063965E-15));
#132073=DIRECTION('center_axis',(-2.35041809182734E-16,-7.08761003338124E-15,
1.));
#132074=DIRECTION('ref_axis',(-1.,1.64128818121889E-30,-2.35041809182734E-16));
#132075=DIRECTION('',(-0.669130606358852,-0.7431448254774,-5.42439438960709E-15));
#132076=DIRECTION('center_axis',(2.35041809182734E-16,7.08761003338124E-15,
-1.));
#132077=DIRECTION('ref_axis',(-1.,-3.73923114693753E-12,-2.35041809209237E-16));
#132078=DIRECTION('',(0.669130606358852,0.7431448254774,5.42439438960709E-15));
#132079=DIRECTION('center_axis',(-2.35041809182734E-16,-7.08761003338124E-15,
1.));
#132080=DIRECTION('ref_axis',(-1.,1.67007359059941E-30,-2.35041809182734E-16));
#132081=DIRECTION('center_axis',(-0.7431448254774,0.669130606358852,4.56786669500647E-15));
#132082=DIRECTION('ref_axis',(2.35041809182734E-16,7.08761003338124E-15,
-1.));
#132083=DIRECTION('center_axis',(-0.743144825477404,0.669130606358847,-1.40595023350398E-14));
#132084=DIRECTION('ref_axis',(0.585256059268642,0.649992703803378,-0.484752338923407));
#132085=DIRECTION('',(0.354588842120041,0.393810805677326,-0.848044693619236));
#132086=DIRECTION('',(-0.669130606358852,-0.7431448254774,-5.42439438960709E-15));
#132087=DIRECTION('',(0.354588491315847,0.393810416069763,0.848045021223114));
#132088=DIRECTION('center_axis',(-0.743144825477429,0.66913060635882,8.60110927597638E-14));
#132089=DIRECTION('ref_axis',(0.585254804454311,0.649991310190875,0.484755722544352));
#132090=DIRECTION('',(0.669130606358852,0.7431448254774,5.28357748271718E-15));
#132091=DIRECTION('',(0.334568657340462,0.371576137911927,-0.866022509672732));
#132092=DIRECTION('center_axis',(0.743144191919631,-0.669131309993359,-1.63998881333916E-6));
#132093=DIRECTION('ref_axis',(0.579515507437722,0.643617174848766,-0.499918702269571));
#132094=DIRECTION('',(0.669130606358852,0.7431448254774,5.28357748271718E-15));
#132095=DIRECTION('center_axis',(0.743145459092284,-0.669129902655552,-1.64014391615252E-6));
#132096=DIRECTION('ref_axis',(0.579496068081958,0.643595585590597,0.499969028326603));
#132097=DIRECTION('',(0.334568762114155,0.371576254274896,0.866022419268947));
#132098=DIRECTION('',(0.669130606358852,0.7431448254774,5.28357748271718E-15));
#132099=DIRECTION('center_axis',(-0.7431448254774,0.669130606358852,4.56786669500647E-15));
#132100=DIRECTION('ref_axis',(2.35041809182734E-16,7.08761003338124E-15,
-1.));
#132101=DIRECTION('center_axis',(0.743144825477371,-0.669130606358884,6.75407619348659E-14));
#132102=DIRECTION('ref_axis',(0.585254804443047,0.649991310178362,0.484755722574728));
#132103=DIRECTION('',(-0.354588491315845,-0.393810416069762,-0.848045021223115));
#132104=DIRECTION('',(0.669130606358852,0.7431448254774,5.42439438960709E-15));
#132105=DIRECTION('',(-0.35458884212002,-0.393810805677306,0.848044693619254));
#132106=DIRECTION('center_axis',(0.743144825477417,-0.669130606358833,-2.48108864766668E-15));
#132107=DIRECTION('ref_axis',(0.585256059282077,0.649992703818338,-0.484752338887127));
#132108=DIRECTION('',(-0.669130606358852,-0.7431448254774,-5.28357748271718E-15));
#132109=DIRECTION('',(-0.334568762114151,-0.371576254274926,-0.866022419268936));
#132110=DIRECTION('center_axis',(-0.743144191772371,0.669131310156907,-1.64037037088548E-6));
#132111=DIRECTION('ref_axis',(0.579515576147878,0.643617251158763,0.499918524374553));
#132112=DIRECTION('',(-0.669130606358852,-0.7431448254774,-5.28357748271718E-15));
#132113=DIRECTION('center_axis',(-0.743145458950891,0.669129902812586,-1.63977760425555E-6));
#132114=DIRECTION('ref_axis',(0.579495997016653,0.643595506664192,-0.499969212295455));
#132115=DIRECTION('',(-0.334568657340465,-0.371576137911891,0.866022509672746));
#132116=DIRECTION('',(-0.669130606358852,-0.7431448254774,-5.28357748271718E-15));
#132117=DIRECTION('center_axis',(-2.23587008033241E-16,-7.09688594845552E-15,
1.));
#132118=DIRECTION('ref_axis',(-1.,1.56129973231166E-30,-2.23587008033241E-16));
#132119=DIRECTION('',(-0.587785252292466,-0.809016994374953,-5.87292248536745E-15));
#132120=DIRECTION('center_axis',(2.23587008033241E-16,7.09688594845552E-15,
-1.));
#132121=DIRECTION('ref_axis',(-1.,-1.22390986234677E-12,-2.23587008041927E-16));
#132122=DIRECTION('',(0.587785252292466,0.809016994374953,5.87292248536745E-15));
#132123=DIRECTION('center_axis',(-2.23587008033241E-16,-7.09688594845552E-15,
1.));
#132124=DIRECTION('ref_axis',(-1.,1.69306078464668E-30,-2.23587008033241E-16));
#132125=DIRECTION('center_axis',(-0.809016994374953,0.587785252292466,3.99055920848344E-15));
#132126=DIRECTION('ref_axis',(2.23587008033241E-16,7.09688594845552E-15,
-1.));
#132127=DIRECTION('center_axis',(-0.809016994374927,0.587785252292501,5.81677449547707E-14));
#132128=DIRECTION('ref_axis',(0.514107226876486,0.707607892256365,-0.484752338921509));
#132129=DIRECTION('',(0.311481929006018,0.428718095637389,-0.848044693619234));
#132130=DIRECTION('',(-0.587785252292466,-0.809016994374953,-5.87292248536745E-15));
#132131=DIRECTION('',(0.31148162084863,0.42871767149512,0.848045021223114));
#132132=DIRECTION('center_axis',(-0.809016994374974,0.587785252292436,5.48596392922833E-14));
#132133=DIRECTION('ref_axis',(0.514106124607928,0.707606375113875,0.484755722543654));
#132134=DIRECTION('',(0.587785252292466,0.809016994374953,5.73210557847754E-15));
#132135=DIRECTION('',(0.29389557254618,0.404512552559094,-0.866022509672745));
#132136=DIRECTION('center_axis',(0.809016437837696,-0.587786018297234,-1.63998882728232E-6));
#132137=DIRECTION('ref_axis',(0.509064546633409,0.700667238055409,-0.499918702267405));
#132138=DIRECTION('',(0.587785252292466,0.809016994374953,5.73210557847754E-15));
#132139=DIRECTION('center_axis',(0.809017550961834,-0.587784486213294,-1.64014398879267E-6));
#132140=DIRECTION('ref_axis',(0.509047470456847,0.700643735094558,0.499969028334988));
#132141=DIRECTION('',(0.293895664582671,0.404512679236444,0.866022419268961));
#132142=DIRECTION('',(0.587785252292466,0.809016994374953,5.73210557847754E-15));
#132143=DIRECTION('center_axis',(-0.809016994374953,0.587785252292466,3.99055920848344E-15));
#132144=DIRECTION('ref_axis',(2.23587008033241E-16,7.09688594845552E-15,
-1.));
#132145=DIRECTION('center_axis',(0.809016994374949,-0.587785252292471,-6.67137321968949E-14));
#132146=DIRECTION('ref_axis',(0.514106124598043,0.707606375100197,0.484755722574104));
#132147=DIRECTION('',(-0.311481620848613,-0.428717671495125,-0.848045021223118));
#132148=DIRECTION('',(0.587785252292466,0.809016994374953,5.87292248536745E-15));
#132149=DIRECTION('',(-0.311481929006028,-0.428718095637371,0.84804469361924));
#132150=DIRECTION('center_axis',(0.809016994374952,-0.587785252292467,-5.23785381174101E-15));
#132151=DIRECTION('ref_axis',(0.514107226887492,0.707607892271531,-0.484752338887699));
#132152=DIRECTION('',(-0.587785252292466,-0.809016994374953,-5.73210557847754E-15));
#132153=DIRECTION('',(-0.293895664582653,-0.404512679236455,-0.866022419268962));
#132154=DIRECTION('center_axis',(-0.809016437708337,0.58778601847528,-1.6403704173616E-6));
#132155=DIRECTION('ref_axis',(0.509064606990258,0.700667321129096,0.499918524373354));
#132156=DIRECTION('',(-0.587785252292466,-0.809016994374953,-5.73210557847754E-15));
#132157=DIRECTION('center_axis',(-0.809017550837597,0.587784486384294,-1.63977757327168E-6));
#132158=DIRECTION('ref_axis',(0.50904740803245,0.700643649174308,-0.49996921229927));
#132159=DIRECTION('',(-0.293895572546189,-0.404512552559082,0.866022509672747));
#132160=DIRECTION('',(-0.587785252292466,-0.809016994374953,-5.73210557847754E-15));
#132161=DIRECTION('center_axis',(-2.11225360334865E-16,-7.10491369633528E-15,
1.));
#132162=DIRECTION('ref_axis',(-1.,1.47497880779919E-30,-2.11225360334865E-16));
#132163=DIRECTION('',(-0.499999999999992,-0.866025403784443,-6.25864843288981E-15));
#132164=DIRECTION('center_axis',(2.11225360334865E-16,7.10491369633528E-15,
-1.));
#132165=DIRECTION('ref_axis',(-1.,-2.39808173319034E-12,-2.11225360351903E-16));
#132166=DIRECTION('',(0.499999999999992,0.866025403784443,6.25864843288981E-15));
#132167=DIRECTION('center_axis',(-2.11225360334865E-16,-7.10491369633528E-15,
1.));
#132168=DIRECTION('ref_axis',(-1.,1.65745742556672E-30,-2.11225360334865E-16));
#132169=DIRECTION('center_axis',(-0.866025403784443,0.499999999999992,3.36953032019407E-15));
#132170=DIRECTION('ref_axis',(2.11225360334864E-16,7.10491369633528E-15,
-1.));
#132171=DIRECTION('center_axis',(-0.866025403784449,0.499999999999982,-2.67406220882125E-14));
#132172=DIRECTION('ref_axis',(0.437325728122339,0.757470380564956,-0.484752338920655));
#132173=DIRECTION('',(0.264962354696012,0.458928260426602,-0.848044693619244));
#132174=DIRECTION('',(-0.499999999999992,-0.866025403784443,-6.25864843288981E-15));
#132175=DIRECTION('',(0.264962092561693,0.458927806396623,0.848045021223114));
#132176=DIRECTION('center_axis',(-0.866025403784433,0.500000000000009,-2.35703475351279E-14));
#132177=DIRECTION('ref_axis',(0.437324790476303,0.757468756514376,0.484755722544276));
#132178=DIRECTION('',(0.499999999999992,0.866025403784443,6.1178315259999E-15));
#132179=DIRECTION('',(0.250002506357492,0.433017043030775,-0.866022509672731));
#132180=DIRECTION('center_axis',(0.866024930365251,-0.500000819982501,-1.6399888658402E-6));
#132181=DIRECTION('ref_axis',(0.433036168125916,0.750040644375568,-0.499918702270186));
#132182=DIRECTION('',(0.499999999999992,0.866025403784443,6.1178315259999E-15));
#132183=DIRECTION('center_axis',(0.866025877245173,-0.499999179938366,-1.64014390875047E-6));
#132184=DIRECTION('ref_axis',(0.433021642224328,0.750015485222473,0.499969028332601));
#132185=DIRECTION('',(0.250002584648419,0.433017178634634,0.866022419268931));
#132186=DIRECTION('',(0.499999999999992,0.866025403784443,6.1178315259999E-15));
#132187=DIRECTION('center_axis',(-0.866025403784443,0.499999999999992,3.36953032019407E-15));
#132188=DIRECTION('ref_axis',(2.11225360334864E-16,7.10491369633528E-15,
-1.));
#132189=DIRECTION('center_axis',(0.866025403784431,-0.500000000000014,5.26542266512672E-14));
#132190=DIRECTION('ref_axis',(0.437324790467692,0.757468756499479,0.484755722575321));
#132191=DIRECTION('',(-0.264962092561685,-0.458927806396634,-0.848045021223111));
#132192=DIRECTION('',(0.499999999999992,0.866025403784443,6.25864843288981E-15));
#132193=DIRECTION('',(-0.264962354696017,-0.458928260426612,0.848044693619237));
#132194=DIRECTION('center_axis',(0.866025403784443,-0.499999999999993,-1.46108553695935E-14));
#132195=DIRECTION('ref_axis',(0.437325728131572,0.757470380580965,-0.484752338887311));
#132196=DIRECTION('',(-0.499999999999992,-0.866025403784443,-6.1178315259999E-15));
#132197=DIRECTION('',(-0.250002584648408,-0.43301717863458,-0.866022419268961));
#132198=DIRECTION('center_axis',(-0.866024930255216,0.500000820173085,-1.6403704313039E-6));
#132199=DIRECTION('ref_axis',(0.433036219468537,0.75004073330313,0.499918524376223));
#132200=DIRECTION('',(-0.499999999999992,-0.866025403784443,-6.1178315259999E-15));
#132201=DIRECTION('center_axis',(-0.86602587713954,0.499999180121329,-1.63977762973091E-6));
#132202=DIRECTION('ref_axis',(0.433021589123383,0.75001539324846,-0.499969212295536));
#132203=DIRECTION('',(-0.25000250635749,-0.433017043030736,0.866022509672752));
#132204=DIRECTION('',(-0.499999999999992,-0.866025403784443,-6.1178315259999E-15));
#132205=DIRECTION('center_axis',(-1.98092302886629E-16,-7.11160532333482E-15,
1.));
#132206=DIRECTION('ref_axis',(-1.,1.38327115779425E-30,-1.98092302886629E-16));
#132207=DIRECTION('',(-0.406736643075792,-0.913545457642605,-6.57734613797476E-15));
#132208=DIRECTION('center_axis',(1.98092302886629E-16,7.11160532333483E-15,
-1.));
#132209=DIRECTION('ref_axis',(-1.,7.04858393874019E-12,-1.98092302836502E-16));
#132210=DIRECTION('',(0.406736643075792,0.913545457642605,6.57734613797476E-15));
#132211=DIRECTION('center_axis',(-1.98092302886629E-16,-7.11160532333483E-15,
1.));
#132212=DIRECTION('ref_axis',(-1.,1.25091873609706E-30,-1.98092302886629E-16));
#132213=DIRECTION('center_axis',(-0.913545457642605,0.406736643075792,2.7115841525971E-15));
#132214=DIRECTION('ref_axis',(1.98092302886629E-16,7.11160532333483E-15,
-1.));
#132215=DIRECTION('center_axis',(-0.913545457642619,0.40673664307576,-5.01731259799456E-14));
#132216=DIRECTION('ref_axis',(0.355752797174364,0.799033864872945,-0.484752338920422));
#132217=DIRECTION('',(0.215539797381043,0.484110311157684,-0.848044693619239));
#132218=DIRECTION('',(-0.406736643075792,-0.913545457642605,-6.57734613797476E-15));
#132219=DIRECTION('',(0.215539584141762,0.484109832214418,0.848045021223121));
#132220=DIRECTION('center_axis',(-0.91354545764262,0.406736643075758,4.31433846695598E-14));
#132221=DIRECTION('ref_axis',(0.3557520344243,0.799032151708265,0.484755722544285));
#132222=DIRECTION('',(0.406736643075792,0.913545457642605,6.43652923108485E-15));
#132223=DIRECTION('',(0.203370360392767,0.456777308164318,-0.866022509672743));
#132224=DIRECTION('center_axis',(0.913545072528379,-0.406737508052096,-1.63998882728247E-6));
#132225=DIRECTION('ref_axis',(0.352263354743371,0.791196448442592,-0.499918702267453));
#132226=DIRECTION('',(0.406736643075792,0.913545457642605,6.43652923108485E-15));
#132227=DIRECTION('center_axis',(0.913545842789922,-0.406735778016344,-1.64014405075982E-6));
#132228=DIRECTION('ref_axis',(0.352251538263023,0.791169908742036,0.499969028333208));
#132229=DIRECTION('',(0.203370424080327,0.456777451208974,0.866022419268936));
#132230=DIRECTION('',(0.406736643075792,0.913545457642605,6.43652923108485E-15));
#132231=DIRECTION('center_axis',(-0.913545457642605,0.406736643075792,2.7115841525971E-15));
#132232=DIRECTION('ref_axis',(1.98092302886629E-16,7.11160532333483E-15,
-1.));
#132233=DIRECTION('center_axis',(0.91354545764259,-0.406736643075824,5.29299032305874E-14));
#132234=DIRECTION('ref_axis',(0.35575203441772,0.799032151693445,0.484755722573542));
#132235=DIRECTION('',(-0.215539584141762,-0.484109832214432,-0.848045021223113));
#132236=DIRECTION('',(0.406736643075792,0.913545457642605,6.57734613797476E-15));
#132237=DIRECTION('',(-0.215539797381046,-0.484110311157701,0.848044693619229));
#132238=DIRECTION('center_axis',(0.913545457642612,-0.406736643075775,7.99461897581586E-15));
#132239=DIRECTION('ref_axis',(0.355752797181782,0.799033864889621,-0.484752338887492));
#132240=DIRECTION('',(-0.406736643075792,-0.913545457642605,-6.43652923108485E-15));
#132241=DIRECTION('',(-0.203370424080328,-0.456777451208907,-0.866022419268971));
#132242=DIRECTION('center_axis',(-0.913545072438836,0.406737508253211,-1.64037047915676E-6));
#132243=DIRECTION('ref_axis',(0.352263396508425,0.791196542247804,0.49991852437719));
#132244=DIRECTION('',(-0.406736643075792,-0.913545457642605,-6.43652923108485E-15));
#132245=DIRECTION('center_axis',(-0.913545842703917,0.406735778209517,-1.63977747463982E-6));
#132246=DIRECTION('ref_axis',(0.352251495066873,0.791169811721274,-0.499969212296194));
#132247=DIRECTION('',(-0.203370360392765,-0.456777308164279,0.866022509672763));
#132248=DIRECTION('',(-0.406736643075792,-0.913545457642605,-6.43652923108485E-15));
#132249=DIRECTION('center_axis',(-1.84331724214206E-16,-7.11688751458844E-15,
1.));
#132250=DIRECTION('ref_axis',(-1.,1.28718155050136E-30,-1.84331724214206E-16));
#132251=DIRECTION('',(-0.309016994374938,-0.951056516295157,-6.82552388187361E-15));
#132252=DIRECTION('center_axis',(1.84331724214206E-16,7.11688751458844E-15,
-1.));
#132253=DIRECTION('ref_axis',(-1.,9.20508114177209E-12,-1.84331724148695E-16));
#132254=DIRECTION('',(0.309016994374938,0.951056516295157,6.82552388187361E-15));
#132255=DIRECTION('center_axis',(-1.84331724214206E-16,-7.11688751458844E-15,
1.));
#132256=DIRECTION('ref_axis',(-1.,1.25755986889655E-30,-1.84331724214206E-16));
#132257=DIRECTION('center_axis',(-0.951056516295157,0.309016994374938,2.0239293015888E-15));
#132258=DIRECTION('ref_axis',(1.84331724214206E-16,7.11688751458845E-15,
-1.));
#132259=DIRECTION('center_axis',(-0.951056516295153,0.309016994374948,8.13245723301314E-15));
#132260=DIRECTION('ref_axis',(0.270282164133991,0.831842966947295,-0.484752338923049));
#132261=DIRECTION('',(0.163755740941343,0.503988348013141,-0.848044693619232));
#132262=DIRECTION('',(-0.309016994374938,-0.951056516295157,-6.82552388187361E-15));
#132263=DIRECTION('',(0.163755578933418,0.503987849403977,0.848045021223128));
#132264=DIRECTION('center_axis',(-0.951056516295156,0.309016994374941,-7.16759106331355E-15));
#132265=DIRECTION('ref_axis',(0.27028158463749,0.831841183440473,0.484755722543016));
#132266=DIRECTION('',(0.309016994374938,0.951056516295157,6.68470697498369E-15));
#132267=DIRECTION('',(0.154510046201588,0.475533025522851,-0.866022509672738));
#132268=DIRECTION('center_axis',(0.95105622370527,-0.309017894868213,-1.63998879715887E-6));
#132269=DIRECTION('ref_axis',(0.267631070329315,0.82368373864957,-0.499918702269331));
#132270=DIRECTION('',(0.309016994374938,0.951056516295157,6.68470697498369E-15));
#132271=DIRECTION('center_axis',(0.951056808909267,-0.309016093795505,-1.6401440671127E-6));
#132272=DIRECTION('ref_axis',(0.26762209273496,0.823656109177694,0.499969028335178));
#132273=DIRECTION('',(0.154510094588028,0.475533174441037,0.86602241926894));
#132274=DIRECTION('',(0.309016994374938,0.951056516295157,6.68470697498369E-15));
#132275=DIRECTION('center_axis',(-0.951056516295157,0.309016994374938,2.0239293015888E-15));
#132276=DIRECTION('ref_axis',(1.84331724214206E-16,7.11688751458845E-15,
-1.));
#132277=DIRECTION('center_axis',(0.951056516295164,-0.309016994374915,-2.46730538496772E-14));
#132278=DIRECTION('ref_axis',(0.270281584632031,0.831841183423701,0.484755722574839));
#132279=DIRECTION('',(-0.163755578933423,-0.503987849403986,-0.848045021223121));
#132280=DIRECTION('',(0.309016994374938,0.951056516295157,6.82552388187361E-15));
#132281=DIRECTION('',(-0.163755740941338,-0.503988348013147,0.84804469361923));
#132282=DIRECTION('center_axis',(0.951056516295147,-0.309016994374969,-4.41082426251915E-14));
#132283=DIRECTION('ref_axis',(0.270282164139995,0.831842966965768,-0.484752338888003));
#132284=DIRECTION('',(-0.309016994374938,-0.951056516295157,-6.68470697498369E-15));
#132285=DIRECTION('',(-0.154510094588046,-0.475533174441003,-0.866022419268957));
#132286=DIRECTION('center_axis',(-0.951056223637252,0.309017895077548,-1.64037042622575E-6));
#132287=DIRECTION('ref_axis',(0.267631102060857,0.823683836308454,0.499918524375601));
#132288=DIRECTION('',(-0.309016994374938,-0.951056516295157,-6.68470697498369E-15));
#132289=DIRECTION('center_axis',(-0.951056808843968,0.309016093996475,-1.63977771355912E-6));
#132290=DIRECTION('ref_axis',(0.267622059916434,0.823656008171873,-0.499969212300578));
#132291=DIRECTION('',(-0.154510046201585,-0.475533025522849,0.866022509672739));
#132292=DIRECTION('',(-0.309016994374938,-0.951056516295157,-6.68470697498369E-15));
#132293=DIRECTION('center_axis',(-1.70094388097117E-16,-7.12070239730339E-15,
1.));
#132294=DIRECTION('ref_axis',(-1.,1.18776276376605E-30,-1.70094388097117E-16));
#132295=DIRECTION('',(-0.207911690817749,-0.978147600733808,-7.00046257728966E-15));
#132296=DIRECTION('center_axis',(1.70094388097117E-16,7.12070239730339E-15,
-1.));
#132297=DIRECTION('ref_axis',(-1.,6.75992595233765E-12,-1.70094388048982E-16));
#132298=DIRECTION('',(0.207911690817749,0.978147600733808,7.00046257728966E-15));
#132299=DIRECTION('center_axis',(-1.70094388097117E-16,-7.12070239730339E-15,
1.));
#132300=DIRECTION('ref_axis',(-1.,1.26081367981038E-30,-1.70094388097117E-16));
#132301=DIRECTION('center_axis',(-0.978147600733808,0.207911690817749,1.31409985761787E-15));
#132302=DIRECTION('ref_axis',(1.70094388097117E-16,7.12070239730339E-15,
-1.));
#132303=DIRECTION('center_axis',(-0.97814760073381,0.20791169081774,-1.98487091788782E-14));
#132304=DIRECTION('ref_axis',(0.181850263143551,0.855538223401766,-0.484752338924911));
#132305=DIRECTION('',(0.110177542335804,0.518344583061406,-0.848044693619233));
#132306=DIRECTION('',(-0.207911690817749,-0.978147600733808,-7.00046257728966E-15));
#132307=DIRECTION('',(0.110177433334219,0.518344070249258,0.848045021223117));
#132308=DIRECTION('center_axis',(-0.97814760073381,0.20791169081774,1.2750041795317E-14));
#132309=DIRECTION('ref_axis',(0.181849873248917,0.85553638909175,0.484755722544049));
#132310=DIRECTION('',(0.207911690817749,0.978147600733808,6.85964567039975E-15));
#132311=DIRECTION('',(0.10395688761095,0.489078703542044,-0.866022509672744));
#132312=DIRECTION('center_axis',(0.978147403873936,-0.207912616962005,-1.63998886076217E-6));
#132313=DIRECTION('ref_axis',(0.180066563904181,0.84714657745213,-0.499918702265563));
#132314=DIRECTION('',(0.207911690817749,0.978147600733808,6.85964567039975E-15));
#132315=DIRECTION('center_axis',(0.978147797608756,-0.207910764585316,-1.64014401168594E-6));
#132316=DIRECTION('ref_axis',(0.180060523556231,0.847118160922957,0.499969028331919));
#132317=DIRECTION('',(0.103956920166113,0.48907885670218,0.866022419268962));
#132318=DIRECTION('',(0.207911690817749,0.978147600733808,6.85964567039975E-15));
#132319=DIRECTION('center_axis',(-0.978147600733808,0.207911690817749,1.31409985761787E-15));
#132320=DIRECTION('ref_axis',(1.70094388097117E-16,7.12070239730339E-15,
-1.));
#132321=DIRECTION('center_axis',(0.97814760073381,-0.207911690817738,-2.52244070083276E-14));
#132322=DIRECTION('ref_axis',(0.181849873245408,0.855536389075222,0.484755722574534));
#132323=DIRECTION('',(-0.110177433334222,-0.518344070249258,-0.848045021223116));
#132324=DIRECTION('',(0.207911690817749,0.978147600733808,7.00046257728966E-15));
#132325=DIRECTION('',(-0.1101775423358,-0.518344583061378,0.848044693619251));
#132326=DIRECTION('center_axis',(0.978147600733805,-0.207911690817764,-2.43284525729549E-14));
#132327=DIRECTION('ref_axis',(0.181850263147838,0.855538223421937,-0.484752338887703));
#132328=DIRECTION('',(-0.207911690817749,-0.978147600733808,-6.85964567039975E-15));
#132329=DIRECTION('',(-0.103956920166104,-0.489078856702181,-0.866022419268962));
#132330=DIRECTION('center_axis',(-0.978147403828179,0.207912617177273,-1.64037039661903E-6));
#132331=DIRECTION('ref_axis',(0.18006658525306,0.847146677889481,0.499918524377841));
#132332=DIRECTION('',(-0.207911690817749,-0.978147600733808,-6.85964567039975E-15));
#132333=DIRECTION('center_axis',(-0.978147797564812,0.207910764792059,-1.63977758902207E-6));
#132334=DIRECTION('ref_axis',(0.180060501475228,0.8471180570388,-0.499969212299415));
#132335=DIRECTION('',(-0.10395688761091,-0.489078703542053,0.866022509672744));
#132336=DIRECTION('',(-0.207911690817749,-0.978147600733808,-6.85964567039975E-15));
#132337=DIRECTION('center_axis',(-1.55536281769216E-16,-7.12300817482632E-15,
1.));
#132338=DIRECTION('ref_axis',(-1.,1.08610405062053E-30,-1.55536281769216E-16));
#132339=DIRECTION('',(-0.104528463267644,-0.994521895368274,-7.10024555926768E-15));
#132340=DIRECTION('center_axis',(1.55536281769216E-16,7.12300817482632E-15,
-1.));
#132341=DIRECTION('ref_axis',(-1.,-2.20623519453511E-12,-1.55536281784931E-16));
#132342=DIRECTION('',(0.104528463267644,0.994521895368274,7.10024555926768E-15));
#132343=DIRECTION('center_axis',(-1.55536281769216E-16,-7.12300817482632E-15,
1.));
#132344=DIRECTION('ref_axis',(-1.,1.26178375522162E-30,-1.55536281769216E-16));
#132345=DIRECTION('center_axis',(-0.994521895368274,0.104528463267644,5.89872860613804E-16));
#132346=DIRECTION('ref_axis',(1.55536281769216E-16,7.12300817482632E-15,
-1.));
#132347=DIRECTION('center_axis',(-0.994521895368273,0.104528463267655,1.83324883388259E-14));
#132348=DIRECTION('ref_axis',(0.0914259726159976,0.869860024050451,-0.484752338921813));
#132349=DIRECTION('',(0.0553922155203034,0.527021726387077,-0.848044693619232));
#132350=DIRECTION('',(-0.104528463267644,-0.994521895368274,-7.10024555926768E-15));
#132351=DIRECTION('',(0.0553921607193071,0.527021204990385,0.848045021223124));
#132352=DIRECTION('center_axis',(-0.994521895368275,0.10452846326764,2.8946040832611E-15));
#132353=DIRECTION('ref_axis',(0.0914257765947068,0.869858159032472,0.484755722543523));
#132354=DIRECTION('',(0.104528463267644,0.994521895368274,6.95942865237777E-15));
#132355=DIRECTION('',(0.0522647556052267,0.49726593293896,-0.86602250967274));
#132356=DIRECTION('center_axis',(0.994521796395256,-0.104529404915857,-1.63998886493578E-6));
#132357=DIRECTION('ref_axis',(0.0905292105226818,0.861327901070913,-0.499918702269594));
#132358=DIRECTION('',(0.104528463267644,0.994521895368274,6.95942865237777E-15));
#132359=DIRECTION('center_axis',(0.994521994347069,-0.104527521530166,-1.64014403561263E-6));
#132360=DIRECTION('ref_axis',(0.090526173600551,0.861299008822545,0.499969028335301));
#132361=DIRECTION('',(0.0522647719724817,0.497266088663029,0.866022419268946));
#132362=DIRECTION('',(0.104528463267644,0.994521895368274,6.95942865237777E-15));
#132363=DIRECTION('center_axis',(-0.994521895368274,0.104528463267644,5.89872860613804E-16));
#132364=DIRECTION('ref_axis',(1.55536281769216E-16,7.12300817482632E-15,
-1.));
#132365=DIRECTION('center_axis',(0.994521895368274,-0.104528463267644,4.4108252692159E-15));
#132366=DIRECTION('ref_axis',(0.0914257765929011,0.869858159015296,0.484755722574685));
#132367=DIRECTION('',(-0.0553921607193093,-0.527021204990427,-0.848045021223098));
#132368=DIRECTION('',(0.104528463267644,0.994521895368274,7.10024555926768E-15));
#132369=DIRECTION('',(-0.0553922155203026,-0.527021726387058,0.848044693619244));
#132370=DIRECTION('center_axis',(0.994521895368274,-0.104528463267646,-1.82635692119912E-15));
#132371=DIRECTION('ref_axis',(0.0914259726179519,0.869860024069042,-0.484752338888083));
#132372=DIRECTION('',(-0.104528463267644,-0.994521895368274,-6.95942865237777E-15));
#132373=DIRECTION('',(-0.0522647719724786,-0.497266088663041,-0.866022419268939));
#132374=DIRECTION('center_axis',(-0.994521796372249,0.104529405134747,-1.64037045376714E-6));
#132375=DIRECTION('ref_axis',(0.0905292212561143,0.861328003190363,0.499918524380586));
#132376=DIRECTION('',(-0.104528463267644,-0.994521895368274,-6.95942865237777E-15));
#132377=DIRECTION('center_axis',(-0.994521994324977,0.104527521740361,-1.63977759371224E-6));
#132378=DIRECTION('ref_axis',(0.0905261624995749,0.861298903201578,-0.499969212298977));
#132379=DIRECTION('',(-0.0522647556052255,-0.497265932938949,0.866022509672747));
#132380=DIRECTION('',(-0.104528463267644,-0.994521895368274,-6.95942865237777E-15));
#132381=DIRECTION('center_axis',(-1.40816906889909E-16,-7.12377958457618E-15,
1.));
#132382=DIRECTION('ref_axis',(0.,-1.,-7.12377958457618E-15));
#132383=DIRECTION('',(1.04744440165294E-14,-1.,-7.12377958457618E-15));
#132384=DIRECTION('',(-1.04744440165294E-14,1.,7.12377958457618E-15));
#132385=DIRECTION('center_axis',(-1.,-1.04744440165294E-14,-1.40816906889984E-16));
#132386=DIRECTION('ref_axis',(1.40816906889909E-16,7.12377958457618E-15,
-1.));
#132387=DIRECTION('center_axis',(-1.,-1.0218985244156E-14,3.06110401690858E-16));
#132388=DIRECTION('ref_axis',(-9.08643805831693E-15,0.874651456243168,-0.484752338923399));
#132389=DIRECTION('',(-5.41813057753238E-15,0.529924709392063,-0.848044693619232));
#132390=DIRECTION('',(1.04744440165294E-14,-1.,-7.12377958457618E-15));
#132391=DIRECTION('',(-5.6761389882299E-15,0.529924185123394,0.848045021223111));
#132392=DIRECTION('center_axis',(-1.,-1.05374547025195E-14,-1.67445974214903E-16));
#132393=DIRECTION('ref_axis',(-9.29775073408689E-15,0.874649580952949,0.484755722543665));
#132394=DIRECTION('',(-1.04744440165294E-14,1.,6.98296267768627E-15));
#132395=DIRECTION('',(-5.23017107763447E-15,0.500005012715,-0.866022509672741));
#132396=DIRECTION('center_axis',(0.999999999998207,-9.46835243406286E-7,
-1.63998885178633E-6));
#132397=DIRECTION('ref_axis',(1.66712506289619E-10,0.866072335963012,-0.499918702270251));
#132398=DIRECTION('',(-1.04744440165294E-14,1.,6.98296267768627E-15));
#132399=DIRECTION('center_axis',(0.999999999998207,9.46924664504057E-7,
-1.64014405074161E-6));
#132400=DIRECTION('ref_axis',(-5.65192826653378E-11,0.866043284544485,0.499969028336156));
#132401=DIRECTION('',(-5.36780659828028E-15,0.500005169296827,0.866022419268954));
#132402=DIRECTION('',(-1.04744440165294E-14,1.,6.98296267768627E-15));
#132403=DIRECTION('center_axis',(-1.,-1.04744440165294E-14,-1.40816906889984E-16));
#132404=DIRECTION('ref_axis',(1.40816906889909E-16,7.12377958457618E-15,
-1.));
#132405=DIRECTION('center_axis',(1.,1.03422010861309E-14,3.74411322160068E-16));
#132406=DIRECTION('ref_axis',(-9.22729987695407E-15,0.874649580936016,0.484755722574217));
#132407=DIRECTION('',(5.62453772470054E-15,-0.529924185123408,-0.848045021223102));
#132408=DIRECTION('',(-1.04744440165294E-14,1.,7.12377958457618E-15));
#132409=DIRECTION('',(5.41813057753242E-15,-0.529924709392054,0.848044693619238));
#132410=DIRECTION('center_axis',(1.,1.04142386870038E-14,-9.91450061389633E-17));
#132411=DIRECTION('ref_axis',(-9.15688980707246E-15,0.874651456262926,-0.484752338887749));
#132412=DIRECTION('',(1.04744440165294E-14,-1.,-6.98296267768627E-15));
#132413=DIRECTION('',(5.50544266490299E-15,-0.50000516929684,-0.866022419268946));
#132414=DIRECTION('center_axis',(-0.999999999998206,9.47055339204534E-7,
-1.64037042584766E-6));
#132415=DIRECTION('ref_axis',(1.66964440532393E-10,0.866072438648236,0.499918524375621));
#132416=DIRECTION('',(1.04744440165294E-14,-1.,-6.98296267768627E-15));
#132417=DIRECTION('center_axis',(-0.999999999998207,-9.46713291890296E-7,
-1.63977758665962E-6));
#132418=DIRECTION('ref_axis',(-5.62799362796097E-11,0.866043178341318,-0.499969212300586));
#132419=DIRECTION('',(5.09253499664396E-15,-0.500005012714988,0.866022509672748));
#132420=DIRECTION('',(1.04744440165294E-14,-1.,-6.98296267768627E-15));
#132421=DIRECTION('center_axis',(-1.26097532010602E-16,-7.12300817482632E-15,
1.));
#132422=DIRECTION('ref_axis',(0.,-1.,-7.12300817482632E-15));
#132423=DIRECTION('',(0.104528463267664,-0.994521895368272,-7.07080680950905E-15));
#132424=DIRECTION('center_axis',(1.26097532010602E-16,7.12300817482632E-15,
-1.));
#132425=DIRECTION('ref_axis',(1.94422256072357E-12,-1.,-7.12300817482607E-15));
#132426=DIRECTION('',(-0.104528463267664,0.994521895368272,7.07080680950905E-15));
#132427=DIRECTION('center_axis',(-1.26097532010602E-16,-7.12300817482632E-15,
1.));
#132428=DIRECTION('ref_axis',(-4.47664446791214E-34,-1.,-7.12300817482632E-15));
#132429=DIRECTION('center_axis',(-0.994521895368272,-0.104528463267664,
-8.69963854894046E-16));
#132430=DIRECTION('ref_axis',(1.26097532010602E-16,7.12300817482632E-15,
-1.));
#132431=DIRECTION('center_axis',(-0.994521895368272,-0.104528463267665,
-4.06622861650637E-15));
#132432=DIRECTION('ref_axis',(0.0914259726158941,-0.869860024049313,0.484752338923875));
#132433=DIRECTION('',(-0.0553922155203146,0.527021726387062,-0.848044693619241));
#132434=DIRECTION('',(0.104528463267664,-0.994521895368272,-7.07080680950905E-15));
#132435=DIRECTION('',(-0.0553921607193175,0.527021204990389,0.848045021223121));
#132436=DIRECTION('center_axis',(-0.994521895368273,-0.104528463267656,
-1.16128759054646E-14));
#132437=DIRECTION('ref_axis',(0.0914257765946433,-0.869858159031697,-0.484755722544926));
#132438=DIRECTION('',(-0.104528463267664,0.994521895368272,6.92998990261914E-15));
#132439=DIRECTION('',(-0.0522647556052188,0.497265932938934,-0.866022509672756));
#132440=DIRECTION('center_axis',(0.994521994337724,0.104527521619073,-1.63998886545253E-6));
#132441=DIRECTION('ref_axis',(0.0905292101912599,-0.861327901107503,0.49991870226657));
#132442=DIRECTION('',(-0.104528463267664,0.994521895368272,6.92998990261914E-15));
#132443=DIRECTION('center_axis',(0.994521796385909,0.104529405004782,-1.64014405966769E-6));
#132444=DIRECTION('ref_axis',(0.0905261737131075,-0.861299008812068,-0.499969028332969));
#132445=DIRECTION('',(-0.0522647719724914,0.497266088663002,0.86602241926896));
#132446=DIRECTION('',(-0.104528463267664,0.994521895368272,6.92998990261914E-15));
#132447=DIRECTION('center_axis',(-0.994521895368272,-0.104528463267664,
-8.69963854894046E-16));
#132448=DIRECTION('ref_axis',(1.26097532010602E-16,7.12300817482632E-15,
-1.));
#132449=DIRECTION('center_axis',(0.994521895368272,0.104528463267664,5.03109757269921E-15));
#132450=DIRECTION('ref_axis',(0.0914257765928723,-0.86985815901481,-0.484755722575562));
#132451=DIRECTION('',(0.0553921607193168,-0.527021204990422,-0.8480450212231));
#132452=DIRECTION('',(-0.104528463267664,0.994521895368272,7.07080680950905E-15));
#132453=DIRECTION('',(0.0553922155203126,-0.527021726387072,0.848044693619235));
#132454=DIRECTION('center_axis',(0.994521895368273,0.104528463267659,-1.53000466606121E-14));
#132455=DIRECTION('ref_axis',(0.091425972618011,-0.869860024069418,0.484752338887397));
#132456=DIRECTION('',(0.104528463267664,-0.994521895368272,-6.92998990261914E-15));
#132457=DIRECTION('',(0.0522647719724914,-0.497266088663002,-0.86602241926896));
#132458=DIRECTION('center_axis',(-0.994521994360728,-0.104527521400198,
-1.64037039730765E-6));
#132459=DIRECTION('ref_axis',(0.0905292209241536,-0.861328003226653,-0.499918524378176));
#132460=DIRECTION('',(0.104528463267664,-0.994521895368272,-6.92998990261914E-15));
#132461=DIRECTION('center_axis',(-0.994521796408006,-0.104529404794558,
-1.63977757761829E-6));
#132462=DIRECTION('ref_axis',(0.0905261626115233,-0.861298903189835,0.499969212298937));
#132463=DIRECTION('',(0.0522647556052198,-0.497265932938937,0.866022509672754));
#132464=DIRECTION('',(0.104528463267664,-0.994521895368272,-6.92998990261914E-15));
#132465=DIRECTION('center_axis',(-1.11539425682701E-16,-7.12070239730339E-15,
1.));
#132466=DIRECTION('ref_axis',(0.,-1.,-7.12070239730339E-15));
#132467=DIRECTION('',(0.20791169081777,-0.978147600733803,-6.94190761487522E-15));
#132468=DIRECTION('center_axis',(1.11539425682701E-16,7.12070239730339E-15,
-1.));
#132469=DIRECTION('ref_axis',(2.43272069155864E-12,-1.,-7.12070239730312E-15));
#132470=DIRECTION('',(-0.20791169081777,0.978147600733803,6.94190761487522E-15));
#132471=DIRECTION('center_axis',(-1.11539425682701E-16,-7.12070239730339E-15,
1.));
#132472=DIRECTION('ref_axis',(1.66310349712474E-34,-1.,-7.12070239730339E-15));
#132473=DIRECTION('center_axis',(-0.978147600733803,-0.20791169081777,-1.58957929685225E-15));
#132474=DIRECTION('ref_axis',(1.11539425682701E-16,7.12070239730339E-15,
-1.));
#132475=DIRECTION('center_axis',(-0.978147600733804,-0.207911690817767,
1.55757231750933E-14));
#132476=DIRECTION('ref_axis',(0.18185026314356,-0.855538223401705,0.484752338925015));
#132477=DIRECTION('',(-0.110177542335814,0.518344583061392,-0.848044693619241));
#132478=DIRECTION('',(0.20791169081777,-0.978147600733803,-6.94190761487522E-15));
#132479=DIRECTION('',(-0.110177433334236,0.518344070249262,0.848045021223112));
#132480=DIRECTION('center_axis',(-0.978147600733805,-0.207911690817763,
-2.29500752315691E-14));
#132481=DIRECTION('ref_axis',(0.181849873249108,-0.855536389092526,-0.484755722542607));
#132482=DIRECTION('',(-0.20791169081777,0.978147600733803,6.80109070798531E-15));
#132483=DIRECTION('',(-0.103956887610934,0.489078703542018,-0.866022509672761));
#132484=DIRECTION('center_axis',(0.978147797590168,0.207910764672768,-1.63998886205246E-6));
#132485=DIRECTION('ref_axis',(0.180066563578227,-0.847146577522247,0.499918702264151));
#132486=DIRECTION('',(-0.20791169081777,0.978147600733803,6.80109070798531E-15));
#132487=DIRECTION('center_axis',(0.978147403855344,0.20791261704947,-1.64014402984576E-6));
#132488=DIRECTION('ref_axis',(0.180060523666867,-0.847118160899729,-0.49996902833143));
#132489=DIRECTION('',(-0.103956920166131,0.489078856702218,0.866022419268938));
#132490=DIRECTION('',(-0.20791169081777,0.978147600733803,6.80109070798531E-15));
#132491=DIRECTION('center_axis',(-0.978147600733803,-0.20791169081777,-1.58957929685225E-15));
#132492=DIRECTION('ref_axis',(1.11539425682701E-16,7.12070239730339E-15,
-1.));
#132493=DIRECTION('center_axis',(0.9781476007338,0.207911690817786,-3.72163382090113E-14));
#132494=DIRECTION('ref_axis',(0.181849873245312,-0.855536389074707,-0.484755722575481));
#132495=DIRECTION('',(0.110177433334237,-0.518344070249266,-0.848045021223109));
#132496=DIRECTION('',(-0.20791169081777,0.978147600733803,6.94190761487522E-15));
#132497=DIRECTION('',(0.11017754233582,-0.518344583061406,0.848044693619231));
#132498=DIRECTION('center_axis',(0.9781476007338,0.207911690817784,3.30811819688897E-14));
#132499=DIRECTION('ref_axis',(0.181850263147783,-0.855538223421614,0.484752338888293));
#132500=DIRECTION('',(0.20791169081777,-0.978147600733803,-6.80109070798531E-15));
#132501=DIRECTION('',(0.103956920166142,-0.489078856702191,-0.866022419268952));
#132502=DIRECTION('center_axis',(-0.978147797635921,-0.207910764457509,
-1.6403703732092E-6));
#132503=DIRECTION('ref_axis',(0.18006658492685,-0.847146677960871,-0.499918524374365));
#132504=DIRECTION('',(0.20791169081777,-0.978147600733803,-6.80109070798531E-15));
#132505=DIRECTION('center_axis',(-0.978147403899293,-0.207912616842712,
-1.63977756346E-6));
#132506=DIRECTION('ref_axis',(0.18006050158514,-0.847118057014537,0.499969212300941));
#132507=DIRECTION('',(0.103956887610927,-0.489078703542022,0.866022509672759));
#132508=DIRECTION('',(0.20791169081777,-0.978147600733803,-6.80109070798531E-15));
#132509=DIRECTION('center_axis',(-9.73020895656121E-17,-7.11688751458844E-15,
1.));
#132510=DIRECTION('ref_axis',(0.,-1.,-7.11688751458844E-15));
#132511=DIRECTION('',(0.309016994374957,-0.95105651629515,-6.73849424722497E-15));
#132512=DIRECTION('center_axis',(9.73020895656121E-17,7.11688751458844E-15,
-1.));
#132513=DIRECTION('ref_axis',(2.04991579266789E-12,-1.,-7.11688751458824E-15));
#132514=DIRECTION('',(-0.309016994374957,0.95105651629515,6.73849424722497E-15));
#132515=DIRECTION('center_axis',(-9.73020895656121E-17,-7.11688751458844E-15,
1.));
#132516=DIRECTION('ref_axis',(-2.26114224696972E-34,-1.,-7.11688751458844E-15));
#132517=DIRECTION('center_axis',(-0.95105651629515,-0.309016994374957,-2.29177897539329E-15));
#132518=DIRECTION('ref_axis',(9.73020895656121E-17,7.11688751458844E-15,
-1.));
#132519=DIRECTION('center_axis',(-0.95105651629515,-0.309016994374959,-2.06757387279998E-14));
#132520=DIRECTION('ref_axis',(0.270282164134165,-0.831842966947816,0.484752338922059));
#132521=DIRECTION('',(-0.163755740941355,0.503988348013135,-0.848044693619233));
#132522=DIRECTION('',(0.309016994374957,-0.95105651629515,-6.73849424722497E-15));
#132523=DIRECTION('',(-0.16375557893343,0.503987849404,0.848045021223112));
#132524=DIRECTION('center_axis',(-0.951056516295154,-0.309016994374946,
-1.50243735750233E-14));
#132525=DIRECTION('ref_axis',(0.270281584637449,-0.831841183440299,-0.484755722543337));
#132526=DIRECTION('',(-0.309016994374957,0.95105651629515,6.59767734033506E-15));
#132527=DIRECTION('',(-0.15451004620158,0.475533025522862,-0.866022509672733));
#132528=DIRECTION('center_axis',(0.951056808881622,0.309016093880587,-1.63998882874534E-6));
#132529=DIRECTION('ref_axis',(0.267631070011315,-0.823683738749887,0.499918702274287));
#132530=DIRECTION('',(-0.309016994374957,0.95105651629515,6.59767734033506E-15));
#132531=DIRECTION('center_axis',(0.951056223677624,0.309017894953297,-1.6401440826045E-6));
#132532=DIRECTION('ref_axis',(0.267622092843495,-0.823656109145871,-0.499969028329508));
#132533=DIRECTION('',(-0.154510094588054,0.475533174441002,0.866022419268955));
#132534=DIRECTION('',(-0.309016994374957,0.95105651629515,6.59767734033506E-15));
#132535=DIRECTION('center_axis',(-0.95105651629515,-0.309016994374957,-2.29177897539329E-15));
#132536=DIRECTION('ref_axis',(9.73020895656121E-17,7.11688751458844E-15,
-1.));
#132537=DIRECTION('center_axis',(0.951056516295148,0.309016994374965,-3.58379553123804E-15));
#132538=DIRECTION('ref_axis',(0.270281584632359,-0.831841183424602,-0.48475572257311));
#132539=DIRECTION('',(0.163755578933425,-0.503987849403991,-0.848045021223118));
#132540=DIRECTION('',(-0.309016994374957,0.95105651629515,6.73849424722497E-15));
#132541=DIRECTION('',(0.16375574094136,-0.503988348013125,0.848044693619238));
#132542=DIRECTION('center_axis',(0.951056516295157,0.309016994374937,-1.84703265992951E-14));
#132543=DIRECTION('ref_axis',(0.27028216414019,-0.831842966966363,0.484752338886874));
#132544=DIRECTION('',(0.309016994374957,-0.95105651629515,-6.59767734033506E-15));
#132545=DIRECTION('',(0.154510094588066,-0.475533174440984,-0.866022419268963));
#132546=DIRECTION('center_axis',(-0.95105680894964,-0.309016093671246,-1.64037039704993E-6));
#132547=DIRECTION('ref_axis',(0.267631101742292,-0.823683836408668,-0.49991852438103));
#132548=DIRECTION('',(0.309016994374957,-0.95105651629515,-6.59767734033506E-15));
#132549=DIRECTION('center_axis',(-0.951056223742958,-0.309017894752224,
-1.63977753144346E-6));
#132550=DIRECTION('ref_axis',(0.267622060023759,-0.823656008137881,0.499969212299128));
#132551=DIRECTION('',(0.154510046201588,-0.475533025522832,0.866022509672748));
#132552=DIRECTION('',(0.309016994374957,-0.95105651629515,-6.59767734033506E-15));
#132553=DIRECTION('center_axis',(-8.35415108931894E-17,-7.11160532333482E-15,
1.));
#132554=DIRECTION('ref_axis',(0.,-1.,-7.11160532333482E-15));
#132555=DIRECTION('',(0.40673664307581,-0.913545457642596,-6.46279534598126E-15));
#132556=DIRECTION('center_axis',(8.35415108931894E-17,7.11160532333482E-15,
-1.));
#132557=DIRECTION('ref_axis',(2.68496336275348E-12,-1.,-7.1116053233346E-15));
#132558=DIRECTION('',(-0.40673664307581,0.913545457642596,6.46279534598126E-15));
#132559=DIRECTION('center_axis',(-8.35415108931894E-17,-7.11160532333482E-15,
1.));
#132560=DIRECTION('ref_axis',(-2.16423649025571E-35,-1.,-7.11160532333482E-15));
#132561=DIRECTION('center_axis',(-0.913545457642596,-0.40673664307581,-2.96886944389434E-15));
#132562=DIRECTION('ref_axis',(8.35415108931894E-17,7.11160532333482E-15,
-1.));
#132563=DIRECTION('center_axis',(-0.913545457642605,-0.40673664307579,5.65136858565243E-14));
#132564=DIRECTION('ref_axis',(0.355752797174256,-0.799033864872624,0.484752338921031));
#132565=DIRECTION('',(-0.215539797381057,0.484110311157699,-0.848044693619227));
#132566=DIRECTION('',(0.40673664307581,-0.913545457642596,-6.46279534598126E-15));
#132567=DIRECTION('',(-0.215539584141776,0.484109832214421,0.848045021223116));
#132568=DIRECTION('center_axis',(-0.913545457642584,-0.406736643075839,
5.12758437606272E-14));
#132569=DIRECTION('ref_axis',(0.355752034424302,-0.799032151708189,-0.484755722544409));
#132570=DIRECTION('',(-0.40673664307581,0.913545457642596,6.32197843909135E-15));
#132571=DIRECTION('',(-0.203370360392764,0.456777308164346,-0.866022509672728));
#132572=DIRECTION('center_axis',(0.913545842753558,0.406735778098021,-1.63998887083193E-6));
#132573=DIRECTION('ref_axis',(0.352263354437923,-0.791196448576317,0.499918702271044));
#132574=DIRECTION('',(-0.40673664307581,0.913545457642596,6.32197843909135E-15));
#132575=DIRECTION('center_axis',(0.913545072492023,0.406737508133752,-1.6401440046282E-6));
#132576=DIRECTION('ref_axis',(0.352251538366133,-0.791169908695755,-0.4999690283338));
#132577=DIRECTION('',(-0.203370424080347,0.456777451208943,0.866022419268948));
#132578=DIRECTION('',(-0.40673664307581,0.913545457642596,6.32197843909135E-15));
#132579=DIRECTION('center_axis',(-0.913545457642596,-0.40673664307581,-2.96886944389434E-15));
#132580=DIRECTION('ref_axis',(8.35415108931894E-17,7.11160532333482E-15,
-1.));
#132581=DIRECTION('center_axis',(0.913545457642598,0.406736643075806,1.40595055456264E-14));
#132582=DIRECTION('ref_axis',(0.355752034418223,-0.799032151694536,-0.484755722571374));
#132583=DIRECTION('',(0.215539584141769,-0.484109832214432,-0.848045021223112));
#132584=DIRECTION('',(-0.40673664307581,0.913545457642596,6.46279534598126E-15));
#132585=DIRECTION('',(0.215539797381038,-0.484110311157674,0.848044693619246));
#132586=DIRECTION('center_axis',(0.913545457642592,0.40673664307582,1.10270606562972E-15));
#132587=DIRECTION('ref_axis',(0.355752797182001,-0.799033864890016,0.484752338886678));
#132588=DIRECTION('',(0.40673664307581,-0.913545457642596,-6.32197843909135E-15));
#132589=DIRECTION('',(0.203370424080339,-0.456777451208961,-0.866022419268941));
#132590=DIRECTION('center_axis',(-0.91354584284308,-0.406735777896949,-1.64037046486974E-6));
#132591=DIRECTION('ref_axis',(0.352263396203447,-0.791196542383823,-0.499918524376819));
#132592=DIRECTION('',(0.40673664307581,-0.913545457642596,-6.32197843909135E-15));
#132593=DIRECTION('center_axis',(-0.913545072577972,-0.406737507940709,
-1.63977757327142E-6));
#132594=DIRECTION('ref_axis',(0.352251495169606,-0.791169811675268,0.499969212296615));
#132595=DIRECTION('',(0.203370360392774,-0.456777308164294,0.866022509672754));
#132596=DIRECTION('',(0.40673664307581,-0.913545457642596,-6.32197843909135E-15));
#132597=DIRECTION('center_axis',(-7.04084534449538E-17,-7.10491369633528E-15,
1.));
#132598=DIRECTION('ref_axis',(0.,-1.,-7.10491369633528E-15));
#132599=DIRECTION('',(0.50000000000001,-0.866025403784433,-6.11783152599983E-15));
#132600=DIRECTION('center_axis',(7.04084534449538E-17,7.10491369633528E-15,
-1.));
#132601=DIRECTION('ref_axis',(3.95505850292466E-12,-1.,-7.104913696335E-15));
#132602=DIRECTION('',(-0.50000000000001,0.866025403784433,6.11783152599983E-15));
#132603=DIRECTION('center_axis',(-7.04084534449538E-17,-7.10491369633528E-15,
1.));
#132604=DIRECTION('ref_axis',(2.79014006612264E-35,-1.,-7.10491369633528E-15));
#132605=DIRECTION('center_axis',(-0.866025403784433,-0.50000000000001,-3.61343235749221E-15));
#132606=DIRECTION('ref_axis',(7.04084534449532E-17,7.10491369633528E-15,
-1.));
#132607=DIRECTION('center_axis',(-0.866025403784415,-0.500000000000041,
-4.57623017179726E-14));
#132608=DIRECTION('ref_axis',(0.437325728121579,-0.75747038056359,0.484752338923477));
#132609=DIRECTION('',(-0.264962354696025,0.458928260426615,-0.848044693619233));
#132610=DIRECTION('',(0.50000000000001,-0.866025403784433,-6.11783152599983E-15));
#132611=DIRECTION('',(-0.264962092561705,0.458927806396624,0.84804502122311));
#132612=DIRECTION('center_axis',(-0.866025403784414,-0.500000000000042,
4.24541932211702E-14));
#132613=DIRECTION('ref_axis',(0.437324790476598,-0.757468756514837,-0.484755722543288));
#132614=DIRECTION('',(-0.50000000000001,0.866025403784433,5.97701461910992E-15));
#132615=DIRECTION('',(-0.250002506357492,0.433017043030769,-0.866022509672735));
#132616=DIRECTION('center_axis',(0.866025877200505,0.499999180015734,-1.63998885826603E-6));
#132617=DIRECTION('ref_axis',(0.433036167836874,-0.750040644541799,0.499918702271157));
#132618=DIRECTION('',(-0.50000000000001,0.866025403784433,5.97701461910992E-15));
#132619=DIRECTION('center_axis',(0.866024930320558,0.500000820059909,-1.64014405299743E-6));
#132620=DIRECTION('ref_axis',(0.433021642322225,-0.750015485165992,-0.49996902833254));
#132621=DIRECTION('',(-0.25000258464842,0.4330171786346,0.866022419268947));
#132622=DIRECTION('',(-0.50000000000001,0.866025403784433,5.97701461910992E-15));
#132623=DIRECTION('center_axis',(-0.866025403784433,-0.50000000000001,-3.61343235749221E-15));
#132624=DIRECTION('ref_axis',(7.04084534449532E-17,7.10491369633528E-15,
-1.));
#132625=DIRECTION('center_axis',(0.866025403784456,0.499999999999971,7.05732043074528E-14));
#132626=DIRECTION('ref_axis',(0.437324790468406,-0.757468756500684,-0.484755722572795));
#132627=DIRECTION('',(0.264962092561699,-0.458927806396623,-0.848045021223113));
#132628=DIRECTION('',(-0.50000000000001,0.866025403784433,6.11783152599983E-15));
#132629=DIRECTION('',(0.264962354696034,-0.45892826042662,0.848044693619228));
#132630=DIRECTION('center_axis',(0.866025403784424,0.500000000000025,2.86703577063736E-14));
#132631=DIRECTION('ref_axis',(0.437325728131524,-0.75747038058083,0.484752338887564));
#132632=DIRECTION('',(0.50000000000001,-0.866025403784433,-5.97701461910992E-15));
#132633=DIRECTION('',(0.250002584648411,-0.433017178634585,-0.866022419268958));
#132634=DIRECTION('center_axis',(-0.866025877310554,-0.499999179825123,
-1.64037042562352E-6));
#132635=DIRECTION('ref_axis',(0.433036219179263,-0.750040733469941,-0.499918524376525));
#132636=DIRECTION('',(0.50000000000001,-0.866025403784433,-5.97701461910992E-15));
#132637=DIRECTION('center_axis',(-0.866024930426216,-0.500000819876906,
-1.63977764694425E-6));
#132638=DIRECTION('ref_axis',(0.433021589220468,-0.750015393191488,0.499969212296916));
#132639=DIRECTION('',(0.25000250635749,-0.433017043030737,0.866022509672751));
#132640=DIRECTION('',(0.50000000000001,-0.866025403784433,-5.97701461910992E-15));
#132641=DIRECTION('center_axis',(-5.80468057465775E-17,-7.09688594845552E-15,
1.));
#132642=DIRECTION('ref_axis',(0.,-1.,-7.09688594845552E-15));
#132643=DIRECTION('',(0.587785252292482,-0.809016994374941,-5.70738228308071E-15));
#132644=DIRECTION('center_axis',(5.80468057465775E-17,7.09688594845552E-15,
-1.));
#132645=DIRECTION('ref_axis',(1.29496413592278E-12,-1.,-7.09688594845544E-15));
#132646=DIRECTION('',(-0.587785252292482,0.809016994374941,5.70738228308071E-15));
#132647=DIRECTION('center_axis',(-5.80468057465775E-17,-7.09688594845552E-15,
1.));
#132648=DIRECTION('ref_axis',(-1.65143981133805E-35,-1.,-7.09688594845552E-15));
#132649=DIRECTION('center_axis',(-0.809016994374941,-0.587785252292482,
-4.21840575002206E-15));
#132650=DIRECTION('ref_axis',(5.80468057465773E-17,7.09688594845552E-15,
-1.));
#132651=DIRECTION('center_axis',(-0.809016994374934,-0.587785252292492,
-1.70919440151463E-14));
#132652=DIRECTION('ref_axis',(0.514107226875991,-0.707607892255666,0.484752338923055));
#132653=DIRECTION('',(-0.311481929006023,0.428718095637386,-0.848044693619234));
#132654=DIRECTION('',(0.587785252292482,-0.809016994374941,-5.70738228308071E-15));
#132655=DIRECTION('',(-0.311481620848639,0.42871767149511,0.848045021223116));
#132656=DIRECTION('center_axis',(-0.809016994374956,-0.587785252292461,
-4.25920315108481E-14));
#132657=DIRECTION('ref_axis',(0.514106124607205,-0.707606375112844,-0.484755722545925));
#132658=DIRECTION('',(-0.587785252292482,0.809016994374941,5.5665653761908E-15));
#132659=DIRECTION('',(-0.293895572546166,0.404512552559088,-0.866022509672753));
#132660=DIRECTION('center_axis',(0.809017550909288,0.587784486285619,-1.6399888522409E-6));
#132661=DIRECTION('ref_axis',(0.509064546362868,-0.700667238250335,0.499918702269694));
#132662=DIRECTION('',(-0.587785252292482,0.809016994374941,5.5665653761908E-15));
#132663=DIRECTION('center_axis',(0.809016437785122,0.587786018369595,-1.64014405557944E-6));
#132664=DIRECTION('ref_axis',(0.509047470547774,-0.700643735027332,-0.499969028336619));
#132665=DIRECTION('',(-0.2938956645827,0.40451267923647,0.866022419268939));
#132666=DIRECTION('',(-0.587785252292482,0.809016994374941,5.5665653761908E-15));
#132667=DIRECTION('center_axis',(-0.809016994374941,-0.587785252292482,
-4.21840575002206E-15));
#132668=DIRECTION('ref_axis',(5.80468057465773E-17,7.09688594845552E-15,
-1.));
#132669=DIRECTION('center_axis',(0.80901699437492,0.587785252292511,-6.86434682521677E-14));
#132670=DIRECTION('ref_axis',(0.514106124598168,-0.707606375100405,-0.484755722573667));
#132671=DIRECTION('',(0.311481620848642,-0.428717671495118,-0.848045021223111));
#132672=DIRECTION('',(-0.587785252292482,0.809016994374941,5.70738228308071E-15));
#132673=DIRECTION('',(0.311481929006041,-0.428718095637379,0.848044693619231));
#132674=DIRECTION('center_axis',(0.809016994374977,0.587785252292433,-9.88300311320588E-14));
#132675=DIRECTION('ref_axis',(0.514107226887611,-0.707607892271672,0.484752338887366));
#132676=DIRECTION('',(0.587785252292482,-0.809016994374941,-5.5665653761908E-15));
#132677=DIRECTION('',(0.293895664582663,-0.404512679236504,-0.866022419268936));
#132678=DIRECTION('center_axis',(-0.809017551038663,-0.587784486107547,
-1.6403705092797E-6));
#132679=DIRECTION('ref_axis',(0.509064606718493,-0.700667321323101,-0.49991852437818));
#132680=DIRECTION('',(0.587785252292482,-0.809016994374941,-5.5665653761908E-15));
#132681=DIRECTION('center_axis',(-0.809016437909362,-0.587786018198594,
-1.63977769066598E-6));
#132682=DIRECTION('ref_axis',(0.509047408122836,-0.700643649107263,0.499969212301199));
#132683=DIRECTION('',(0.293895572546205,-0.40451255255908,0.866022509672743));
#132684=DIRECTION('',(0.587785252292482,-0.809016994374941,-5.5665653761908E-15));
#132685=DIRECTION('center_axis',(-4.65920045970846E-17,-7.08761003338123E-15,
1.));
#132686=DIRECTION('ref_axis',(0.,-1.,-7.08761003338124E-15));
#132687=DIRECTION('',(0.669130606358867,-0.743144825477386,-5.23594458502135E-15));
#132688=DIRECTION('center_axis',(4.65920045970846E-17,7.08761003338124E-15,
-1.));
#132689=DIRECTION('ref_axis',(-5.08215691752411E-12,-1.,-7.08761003338147E-15));
#132690=DIRECTION('',(-0.669130606358867,0.743144825477386,5.23594458502135E-15));
#132691=DIRECTION('center_axis',(-4.65920045970846E-17,-7.08761003338124E-15,
1.));
#132692=DIRECTION('ref_axis',(-1.03129032759636E-34,-1.,-7.08761003338123E-15));
#132693=DIRECTION('center_axis',(-0.743144825477386,-0.669130606358867,
-4.77716140639652E-15));
#132694=DIRECTION('ref_axis',(4.65920045970844E-17,7.08761003338124E-15,
-1.));
#132695=DIRECTION('center_axis',(-0.743144825477404,-0.669130606358848,
1.37838258186658E-14));
#132696=DIRECTION('ref_axis',(0.585256059268725,-0.64999270380347,0.484752338923184));
#132697=DIRECTION('',(-0.354588842120043,0.393810805677302,-0.848044693619246));
#132698=DIRECTION('',(0.669130606358867,-0.743144825477386,-5.23594458502135E-15));
#132699=DIRECTION('',(-0.354588491315847,0.39381041606975,0.84804502122312));
#132700=DIRECTION('center_axis',(-0.743144825477363,-0.669130606358893,
8.68381224978359E-14));
#132701=DIRECTION('ref_axis',(0.585254804454868,-0.649991310191489,-0.484755722542855));
#132702=DIRECTION('',(-0.669130606358867,0.743144825477386,5.09512767813144E-15));
#132703=DIRECTION('',(-0.33456865734045,0.371576137911913,-0.866022509672743));
#132704=DIRECTION('center_axis',(0.743145459032533,0.669129902721913,-1.63998890336437E-6));
#132705=DIRECTION('ref_axis',(0.579515507191614,-0.643617175073762,0.499918702265194));
#132706=DIRECTION('',(-0.669130606358867,0.743144825477386,5.09512767813144E-15));
#132707=DIRECTION('center_axis',(0.743144191859767,0.669131310059845,-1.64014407107154E-6));
#132708=DIRECTION('ref_axis',(0.579496068163303,-0.643595585511986,-0.499969028333513));
#132709=DIRECTION('',(-0.334568762114147,0.371576254274927,0.866022419268937));
#132710=DIRECTION('',(-0.669130606358867,0.743144825477386,5.09512767813144E-15));
#132711=DIRECTION('center_axis',(-0.743144825477386,-0.669130606358867,
-4.77716140639652E-15));
#132712=DIRECTION('ref_axis',(4.65920045970844E-17,7.08761003338124E-15,
-1.));
#132713=DIRECTION('center_axis',(0.743144825477406,0.669130606358846,1.31773404917825E-13));
#132714=DIRECTION('ref_axis',(0.585254804442819,-0.649991310178033,-0.484755722575444));
#132715=DIRECTION('',(0.35458849131585,-0.393810416069767,-0.848045021223111));
#132716=DIRECTION('',(-0.669130606358867,0.743144825477386,5.23594458502135E-15));
#132717=DIRECTION('',(0.354588842120061,-0.393810805677319,0.848044693619231));
#132718=DIRECTION('center_axis',(0.743144825477364,0.669130606358892,1.20746314186455E-13));
#132719=DIRECTION('ref_axis',(0.585256059281856,-0.649992703818073,0.48475233888775));
#132720=DIRECTION('',(0.669130606358867,-0.743144825477386,-5.09512767813144E-15));
#132721=DIRECTION('',(0.334568762114181,-0.371576254274921,-0.866022419268926));
#132722=DIRECTION('center_axis',(-0.743145459179761,-0.669129902558398,
-1.64037041512388E-6));
#132723=DIRECTION('ref_axis',(0.579515575899139,-0.643617251381538,-0.499918524376086));
#132724=DIRECTION('',(0.669130606358867,-0.743144825477386,-5.09512767813144E-15));
#132725=DIRECTION('center_axis',(-0.743144192001212,-0.669131309902755,
-1.63977757292739E-6));
#132726=DIRECTION('ref_axis',(0.579495997099853,-0.643595506588377,0.499969212296615));
#132727=DIRECTION('',(0.334568657340469,-0.371576137911896,0.866022509672743));
#132728=DIRECTION('',(0.669130606358867,-0.743144825477386,-5.09512767813144E-15));
#132729=DIRECTION('center_axis',(-3.61695511949404E-17,-7.07718757997909E-15,
1.));
#132730=DIRECTION('ref_axis',(0.,-1.,-7.07718757997909E-15));
#132731=DIRECTION('',(0.743144825477402,-0.66913060635885,-4.70868360189637E-15));
#132732=DIRECTION('center_axis',(3.61695511949404E-17,7.07718757997909E-15,
-1.));
#132733=DIRECTION('ref_axis',(1.24700250125898E-12,-1.,-7.07718757997905E-15));
#132734=DIRECTION('',(-0.743144825477402,0.66913060635885,4.70868360189637E-15));
#132735=DIRECTION('center_axis',(-3.61695511949404E-17,-7.07718757997909E-15,
1.));
#132736=DIRECTION('ref_axis',(7.4438098531367E-35,-1.,-7.07718757997909E-15));
#132737=DIRECTION('center_axis',(-0.66913060635885,-0.743144825477402,-5.2835774827172E-15));
#132738=DIRECTION('ref_axis',(3.61695511949403E-17,7.07718757997909E-15,
-1.));
#132739=DIRECTION('center_axis',(-0.669130606358838,-0.743144825477412,
-6.12001866348751E-14));
#132740=DIRECTION('ref_axis',(0.649992703804337,-0.585256059269522,0.484752338921059));
#132741=DIRECTION('',(-0.393810805677327,0.354588842120035,-0.848044693619238));
#132742=DIRECTION('',(0.743144825477402,-0.66913060635885,-4.70868360189637E-15));
#132743=DIRECTION('',(-0.393810416069782,0.354588491315838,0.848045021223109));
#132744=DIRECTION('center_axis',(-0.669130606358808,-0.743144825477439,
6.53353493078882E-14));
#132745=DIRECTION('ref_axis',(0.649991310191254,-0.58525480445462,-0.484755722543471));
#132746=DIRECTION('',(-0.743144825477402,0.66913060635885,4.56786669500646E-15));
#132747=DIRECTION('',(-0.371576137911926,0.334568657340426,-0.866022509672746));
#132748=DIRECTION('center_axis',(0.669131309993341,0.743144191919648,-1.63998873674059E-6));
#132749=DIRECTION('ref_axis',(0.643617174849297,-0.579515507438223,0.499918702268307));
#132750=DIRECTION('',(-0.743144825477402,0.66913060635885,4.56786669500646E-15));
#132751=DIRECTION('center_axis',(0.669129902655539,0.743145459092296,-1.64014398156296E-6));
#132752=DIRECTION('ref_axis',(0.643595585587785,-0.579496068079448,-0.499969028333132));
#132753=DIRECTION('',(-0.371576254274935,0.334568762114158,0.866022419268929));
#132754=DIRECTION('',(-0.743144825477402,0.66913060635885,4.56786669500646E-15));
#132755=DIRECTION('center_axis',(-0.66913060635885,-0.743144825477402,-5.2835774827172E-15));
#132756=DIRECTION('ref_axis',(3.61695511949403E-17,7.07718757997909E-15,
-1.));
#132757=DIRECTION('center_axis',(0.669130606358883,0.743144825477372,6.25785835070068E-14));
#132758=DIRECTION('ref_axis',(0.649991310179483,-0.585254804444058,-0.484755722572005));
#132759=DIRECTION('',(0.393810416069765,-0.354588491315822,-0.848045021223123));
#132760=DIRECTION('',(-0.743144825477402,0.66913060635885,4.70868360189637E-15));
#132761=DIRECTION('',(0.393810805677295,-0.354588842120035,0.848044693619253));
#132762=DIRECTION('center_axis',(0.669130606358823,0.743144825477426,-4.13514774611113E-15));
#132763=DIRECTION('ref_axis',(0.649992703818683,-0.585256059282372,0.48475233888631));
#132764=DIRECTION('',(0.743144825477402,-0.66913060635885,-4.56786669500646E-15));
#132765=DIRECTION('',(0.371576254274878,-0.334568762114136,-0.866022419268962));
#132766=DIRECTION('center_axis',(-0.669131310156998,-0.743144191772289,
-1.64037057985418E-6));
#132767=DIRECTION('ref_axis',(0.643617251158517,-0.579515576147659,-0.499918524375124));
#132768=DIRECTION('',(0.743144825477402,-0.66913060635885,-4.56786669500646E-15));
#132769=DIRECTION('center_axis',(-0.669129902812614,-0.743145458950866,
-1.63977747515624E-6));
#132770=DIRECTION('ref_axis',(0.643595506663296,-0.579495997015805,0.499969212297591));
#132771=DIRECTION('',(0.371576137911909,-0.334568657340446,0.866022509672746));
#132772=DIRECTION('',(0.743144825477402,-0.66913060635885,-4.56786669500646E-15));
#132773=DIRECTION('center_axis',(-2.68936361206573E-17,-7.0657327788296E-15,
1.));
#132774=DIRECTION('ref_axis',(0.,-1.,-7.0657327788296E-15));
#132775=DIRECTION('',(0.809016994374955,-0.587785252292463,-4.13137611537333E-15));
#132776=DIRECTION('center_axis',(2.68936361206573E-17,7.0657327788296E-15,
-1.));
#132777=DIRECTION('ref_axis',(1.22302168392707E-12,-1.,-7.06573277882956E-15));
#132778=DIRECTION('',(-0.809016994374955,0.587785252292463,4.13137611537333E-15));
#132779=DIRECTION('center_axis',(-2.68936361206573E-17,-7.0657327788296E-15,
1.));
#132780=DIRECTION('ref_axis',(-5.51266204707114E-35,-1.,-7.0657327788296E-15));
#132781=DIRECTION('center_axis',(-0.587785252292463,-0.809016994374955,
-5.73210557847756E-15));
#132782=DIRECTION('ref_axis',(2.68936361206571E-17,7.0657327788296E-15,
-1.));
#132783=DIRECTION('center_axis',(-0.587785252292406,-0.809016994374997,
-1.16611166425919E-13));
#132784=DIRECTION('ref_axis',(0.707607892255381,-0.514107226875749,0.484752338923727));
#132785=DIRECTION('',(-0.428718095637369,0.31148192900601,-0.848044693619247));
#132786=DIRECTION('',(0.809016994374955,-0.587785252292463,-4.13137611537333E-15));
#132787=DIRECTION('',(-0.428717671495122,0.311481620848618,0.848045021223118));
#132788=DIRECTION('center_axis',(-0.587785252292469,-0.809016994374951,
-1.77811393686054E-14));
#132789=DIRECTION('ref_axis',(0.707606375113731,-0.514106124607824,-0.484755722543974));
#132790=DIRECTION('',(-0.809016994374955,0.587785252292463,3.99055920848342E-15));
#132791=DIRECTION('',(-0.404512552559104,0.293895572546187,-0.866022509672738));
#132792=DIRECTION('center_axis',(0.587786018297211,0.809016437837712,-1.63998882504441E-6));
#132793=DIRECTION('ref_axis',(0.700667238053777,-0.509064546632195,0.499918702270929));
#132794=DIRECTION('',(-0.809016994374955,0.587785252292463,3.99055920848342E-15));
#132795=DIRECTION('center_axis',(0.587784486213298,0.809017550961831,-1.64014397261229E-6));
#132796=DIRECTION('ref_axis',(0.700643735093623,-0.509047470456162,-0.499969028336995));
#132797=DIRECTION('',(-0.404512679236441,0.293895664582704,0.866022419268951));
#132798=DIRECTION('',(-0.809016994374955,0.587785252292463,3.99055920848342E-15));
#132799=DIRECTION('center_axis',(-0.587785252292463,-0.809016994374955,
-5.73210557847756E-15));
#132800=DIRECTION('ref_axis',(2.68936361206571E-17,7.0657327788296E-15,
-1.));
#132801=DIRECTION('center_axis',(0.587785252292428,0.80901699437498,-5.15515203339627E-14));
#132802=DIRECTION('ref_axis',(0.707606375100059,-0.514106124597877,-0.48475572257448));
#132803=DIRECTION('',(0.428717671495112,-0.311481620848614,-0.848045021223125));
#132804=DIRECTION('',(-0.809016994374955,0.587785252292463,4.13137611537333E-15));
#132805=DIRECTION('',(0.428718095637375,-0.311481929006031,0.848044693619236));
#132806=DIRECTION('center_axis',(0.587785252292464,0.809016994374954,7.58110420120383E-15));
#132807=DIRECTION('ref_axis',(0.707607892271749,-0.514107226887654,0.484752338887208));
#132808=DIRECTION('',(0.809016994374955,-0.587785252292463,-3.99055920848342E-15));
#132809=DIRECTION('',(0.404512679236445,-0.293895664582672,-0.86602241926896));
#132810=DIRECTION('center_axis',(-0.587786018475315,-0.809016437708311,
-1.64037046349258E-6));
#132811=DIRECTION('ref_axis',(0.700667321127176,-0.509064606988881,-0.499918524377446));
#132812=DIRECTION('',(0.809016994374955,-0.587785252292463,-3.99055920848342E-15));
#132813=DIRECTION('center_axis',(-0.587784486384234,-0.80901755083764,-1.63977767276418E-6));
#132814=DIRECTION('ref_axis',(0.700643649175429,-0.509047408033247,0.499969212296889));
#132815=DIRECTION('',(0.404512552559084,-0.293895572546137,0.866022509672764));
#132816=DIRECTION('',(0.809016994374955,-0.587785252292463,-3.99055920848342E-15));
#132817=DIRECTION('center_axis',(-1.88658882408992E-17,-7.05337113113122E-15,
1.));
#132818=DIRECTION('ref_axis',(0.,-1.,-7.05337113113122E-15));
#132819=DIRECTION('',(0.866025403784445,-0.499999999999989,-3.51034722708395E-15));
#132820=DIRECTION('center_axis',(1.88658882408992E-17,7.05337113113122E-15,
-1.));
#132821=DIRECTION('ref_axis',(1.7245796508144E-35,-1.,-7.05337113113122E-15));
#132822=DIRECTION('',(-0.866025403784445,0.499999999999989,3.51034722708395E-15));
#132823=DIRECTION('center_axis',(-1.88658882408992E-17,-7.05337113113122E-15,
1.));
#132824=DIRECTION('ref_axis',(5.32933612927079E-36,-1.,-7.05337113113122E-15));
#132825=DIRECTION('center_axis',(-0.499999999999989,-0.866025403784445,
-6.11783152599991E-15));
#132826=DIRECTION('ref_axis',(1.88658882408991E-17,7.05337113113122E-15,
-1.));
#132827=DIRECTION('center_axis',(-0.500000000000019,-0.866025403784427,
1.90216796297591E-14));
#132828=DIRECTION('ref_axis',(0.7574703805651,-0.437325728122441,0.484752338920339));
#132829=DIRECTION('',(-0.458928260426615,0.264962354696012,-0.848044693619237));
#132830=DIRECTION('',(0.866025403784445,-0.499999999999989,-3.51034722708395E-15));
#132831=DIRECTION('',(-0.458927806396625,0.264962092561681,0.848045021223117));
#132832=DIRECTION('center_axis',(-0.499999999999992,-0.866025403784443,
4.09379720346935E-14));
#132833=DIRECTION('ref_axis',(0.757468756514768,-0.437324790476546,-0.484755722543443));
#132834=DIRECTION('',(-0.866025403784445,0.499999999999989,3.36953032019404E-15));
#132835=DIRECTION('',(-0.433017043030785,0.250002506357516,-0.86602250967272));
#132836=DIRECTION('center_axis',(0.500000819982458,0.866024930365276,-1.63998880283935E-6));
#132837=DIRECTION('ref_axis',(0.750040644375926,-0.43303616812611,0.49991870226948));
#132838=DIRECTION('',(-0.866025403784445,0.499999999999989,3.36953032019404E-15));
#132839=DIRECTION('center_axis',(0.49999917993825,0.86602587724524,-1.64014411875219E-6));
#132840=DIRECTION('ref_axis',(0.750015485220901,-0.433021642223407,-0.499969028335756));
#132841=DIRECTION('',(-0.433017178634628,0.25000258464838,0.866022419268945));
#132842=DIRECTION('',(-0.866025403784445,0.499999999999989,3.36953032019404E-15));
#132843=DIRECTION('center_axis',(-0.499999999999989,-0.866025403784445,
-6.11783152599991E-15));
#132844=DIRECTION('ref_axis',(1.88658882408991E-17,7.05337113113122E-15,
-1.));
#132845=DIRECTION('center_axis',(0.499999999999992,0.866025403784443,2.56379218773161E-14));
#132846=DIRECTION('ref_axis',(0.757468756499777,-0.437324790467854,-0.48475572257471));
#132847=DIRECTION('',(0.458927806396632,-0.264962092561684,-0.848045021223112));
#132848=DIRECTION('',(-0.866025403784445,0.499999999999989,3.51034722708395E-15));
#132849=DIRECTION('',(0.458928260426591,-0.264962354696007,0.848044693619252));
#132850=DIRECTION('center_axis',(0.499999999999983,0.866025403784448,1.94351944067221E-14));
#132851=DIRECTION('ref_axis',(0.757470380580877,-0.437325728131528,0.484752338887488));
#132852=DIRECTION('',(0.866025403784445,-0.499999999999989,-3.36953032019404E-15));
#132853=DIRECTION('',(0.433017178634599,-0.250002584648384,-0.866022419268958));
#132854=DIRECTION('center_axis',(-0.500000820173042,-0.866024930255241,
-1.64037038534468E-6));
#132855=DIRECTION('ref_axis',(0.750040733305284,-0.433036219469757,-0.499918524371935));
#132856=DIRECTION('',(0.866025403784445,-0.499999999999989,-3.36953032019404E-15));
#132857=DIRECTION('center_axis',(-0.499999180121316,-0.866025877139547,
-1.639777584288E-6));
#132858=DIRECTION('ref_axis',(0.750015393247918,-0.433021589123031,0.499969212296653));
#132859=DIRECTION('',(0.433017043030737,-0.25000250635749,0.866022509672751));
#132860=DIRECTION('',(0.866025403784445,-0.499999999999989,-3.36953032019404E-15));
#132861=DIRECTION('center_axis',(-1.2174261241351E-17,-7.04023807368298E-15,
1.));
#132862=DIRECTION('ref_axis',(0.,-1.,-7.04023807368299E-15));
#132863=DIRECTION('',(0.913545457642606,-0.406736643075789,-2.85240105948698E-15));
#132864=DIRECTION('center_axis',(1.2174261241351E-17,7.04023807368298E-15,
-1.));
#132865=DIRECTION('ref_axis',(-7.04858393874019E-12,-1.,-7.04023807368307E-15));
#132866=DIRECTION('',(-0.913545457642606,0.406736643075789,2.85240105948698E-15));
#132867=DIRECTION('center_axis',(-1.2174261241351E-17,-7.04023807368298E-15,
1.));
#132868=DIRECTION('ref_axis',(2.24415770289596E-35,-1.,-7.04023807368298E-15));
#132869=DIRECTION('center_axis',(-0.406736643075789,-0.913545457642606,
-6.43652923108486E-15));
#132870=DIRECTION('ref_axis',(1.21742612413511E-17,7.04023807368299E-15,
-1.));
#132871=DIRECTION('center_axis',(-0.406736643075775,-0.913545457642612,
-5.54109797910375E-14));
#132872=DIRECTION('ref_axis',(0.799033864872087,-0.355752797174001,0.484752338922104));
#132873=DIRECTION('',(-0.484110311157674,0.215539797381038,-0.848044693619246));
#132874=DIRECTION('',(0.913545457642606,-0.406736643075789,-2.85240105948698E-15));
#132875=DIRECTION('',(-0.484109832214431,0.215539584141763,0.848045021223114));
#132876=DIRECTION('center_axis',(-0.406736643075784,-0.913545457642608,
-1.07513865949709E-14));
#132877=DIRECTION('ref_axis',(0.79903215170898,-0.355752034424618,-0.484755722542873));
#132878=DIRECTION('',(-0.913545457642606,0.406736643075789,2.71158415259707E-15));
#132879=DIRECTION('',(-0.456777308164329,0.203370360392772,-0.866022509672736));
#132880=DIRECTION('center_axis',(0.406737508052128,0.913545072528365,-1.63998884277371E-6));
#132881=DIRECTION('ref_axis',(0.791196448441515,-0.352263354742916,0.499918702269479));
#132882=DIRECTION('',(-0.913545457642606,0.406736643075789,2.71158415259707E-15));
#132883=DIRECTION('center_axis',(0.406735778016422,0.913545842789888,-1.64014388757881E-6));
#132884=DIRECTION('ref_axis',(0.791169908742249,-0.352251538263108,-0.499969028332811));
#132885=DIRECTION('',(-0.456777451208919,0.203370424080316,0.866022419268968));
#132886=DIRECTION('',(-0.913545457642606,0.406736643075789,2.71158415259707E-15));
#132887=DIRECTION('center_axis',(-0.406736643075789,-0.913545457642606,
-6.43652923108486E-15));
#132888=DIRECTION('ref_axis',(1.21742612413511E-17,7.04023807368299E-15,
-1.));
#132889=DIRECTION('center_axis',(0.406736643075769,0.913545457642615,1.24054460696708E-14));
#132890=DIRECTION('ref_axis',(0.79903215169305,-0.355752034417508,-0.484755722574348));
#132891=DIRECTION('',(0.484109832214428,-0.21553958414176,-0.848045021223116));
#132892=DIRECTION('',(-0.913545457642606,0.406736643075789,2.85240105948698E-15));
#132893=DIRECTION('',(0.484110311157676,-0.215539797381039,0.848044693619245));
#132894=DIRECTION('center_axis',(0.406736643075817,0.913545457642593,-4.39704043669829E-14));
#132895=DIRECTION('ref_axis',(0.799033864889077,-0.355752797181557,0.484752338888553));
#132896=DIRECTION('',(0.913545457642606,-0.406736643075789,-2.71158415259707E-15));
#132897=DIRECTION('',(0.456777451208934,-0.203370424080325,-0.866022419268958));
#132898=DIRECTION('center_axis',(-0.406737508253126,-0.913545072438874,
-1.64037033628669E-6));
#132899=DIRECTION('ref_axis',(0.791196542248508,-0.352263396508728,-0.499918524375862));
#132900=DIRECTION('',(0.913545457642606,-0.406736643075789,-2.71158415259707E-15));
#132901=DIRECTION('center_axis',(-0.406735778209486,-0.913545842703931,
-1.63977751199268E-6));
#132902=DIRECTION('ref_axis',(0.791169811719898,-0.352251495066249,0.499969212298812));
#132903=DIRECTION('',(0.456777308164306,-0.203370360392779,0.866022509672746));
#132904=DIRECTION('',(0.913545457642606,-0.406736643075789,-2.71158415259707E-15));
#132905=DIRECTION('center_axis',(-6.89206998773264E-18,-7.02647749501056E-15,
1.));
#132906=DIRECTION('ref_axis',(0.,-1.,-7.02647749501056E-15));
#132907=DIRECTION('',(0.951056516295158,-0.309016994374935,-2.16474620847869E-15));
#132908=DIRECTION('center_axis',(6.89206998773264E-18,7.02647749501056E-15,
-1.));
#132909=DIRECTION('ref_axis',(-6.90292267790937E-12,-1.,-7.02647749501061E-15));
#132910=DIRECTION('',(-0.951056516295158,0.309016994374935,2.16474620847869E-15));
#132911=DIRECTION('center_axis',(-6.89206998773264E-18,-7.02647749501056E-15,
1.));
#132912=DIRECTION('ref_axis',(1.91373385038743E-35,-1.,-7.02647749501056E-15));
#132913=DIRECTION('center_axis',(-0.309016994374935,-0.951056516295158,
-6.6847069749837E-15));
#132914=DIRECTION('ref_axis',(6.89206998773277E-18,7.02647749501056E-15,
-1.));
#132915=DIRECTION('center_axis',(-0.309016994374942,-0.951056516295155,
2.52244012481594E-14));
#132916=DIRECTION('ref_axis',(0.831842966947875,-0.270282164134165,0.484752338921958));
#132917=DIRECTION('',(-0.503988348013123,0.163755740941358,-0.84804469361924));
#132918=DIRECTION('',(0.951056516295158,-0.309016994374935,-2.16474620847869E-15));
#132919=DIRECTION('',(-0.503987849404009,0.163755578933409,0.848045021223111));
#132920=DIRECTION('center_axis',(-0.309016994374912,-0.951056516295165,
4.46596058560273E-14));
#132921=DIRECTION('ref_axis',(0.831841183439677,-0.270281584637229,-0.484755722544527));
#132922=DIRECTION('',(-0.951056516295158,0.309016994374935,2.02392930158878E-15));
#132923=DIRECTION('',(-0.475533025522877,0.154510046201611,-0.866022509672719));
#132924=DIRECTION('center_axis',(0.309017894868202,0.951056223705274,-1.6399888374375E-6));
#132925=DIRECTION('ref_axis',(0.823683738650715,-0.267631070329656,0.499918702267262));
#132926=DIRECTION('',(-0.951056516295158,0.309016994374935,2.02392930158878E-15));
#132927=DIRECTION('center_axis',(0.309016093795519,0.951056808909262,-1.64014404180921E-6));
#132928=DIRECTION('ref_axis',(0.823656109178864,-0.26762209273534,-0.499969028333049));
#132929=DIRECTION('',(-0.475533174441005,0.154510094588011,0.866022419268961));
#132930=DIRECTION('',(-0.951056516295158,0.309016994374935,2.02392930158878E-15));
#132931=DIRECTION('center_axis',(-0.309016994374935,-0.951056516295158,
-6.6847069749837E-15));
#132932=DIRECTION('ref_axis',(6.89206998773277E-18,7.02647749501056E-15,
-1.));
#132933=DIRECTION('center_axis',(0.309016994374906,0.951056516295167,-2.55000835876527E-14));
#132934=DIRECTION('ref_axis',(0.831841183424368,-0.27028158463224,-0.484755722573579));
#132935=DIRECTION('',(0.503987849404013,-0.163755578933417,-0.848045021223107));
#132936=DIRECTION('',(-0.951056516295158,0.309016994374935,2.16474620847869E-15));
#132937=DIRECTION('',(0.503988348013109,-0.163755740941346,0.84804469361925));
#132938=DIRECTION('center_axis',(0.30901699437495,0.951056516295153,-1.10270606562971E-14));
#132939=DIRECTION('ref_axis',(0.831842966967129,-0.270282164140436,0.484752338885422));
#132940=DIRECTION('',(0.951056516295158,-0.309016994374935,-2.02392930158878E-15));
#132941=DIRECTION('',(0.475533174441021,-0.154510094588014,-0.866022419268952));
#132942=DIRECTION('center_axis',(-0.309017895077545,-0.951056223637253,
-1.64037043268108E-6));
#132943=DIRECTION('ref_axis',(0.823683836308317,-0.267631102060807,-0.499918524375855));
#132944=DIRECTION('',(0.951056516295158,-0.309016994374935,-2.02392930158878E-15));
#132945=DIRECTION('center_axis',(-0.309016093996576,-0.951056808843936,
-1.63977750631261E-6));
#132946=DIRECTION('ref_axis',(0.823656008174437,-0.267622059917255,0.499969212295914));
#132947=DIRECTION('',(0.475533025522831,-0.154510046201605,0.866022509672745));
#132948=DIRECTION('',(0.951056516295158,-0.309016994374935,-2.02392930158878E-15));
#132949=DIRECTION('center_axis',(-3.07718727278846E-18,-7.01224015889347E-15,
1.));
#132950=DIRECTION('ref_axis',(0.,-1.,-7.01224015889347E-15));
#132951=DIRECTION('',(0.978147600733808,-0.207911690817747,-1.45491676450776E-15));
#132952=DIRECTION('center_axis',(3.07718727278846E-18,7.01224015889347E-15,
-1.));
#132953=DIRECTION('ref_axis',(2.25419682919892E-12,-1.,-7.01224015889347E-15));
#132954=DIRECTION('',(-0.978147600733808,0.207911690817747,1.45491676450776E-15));
#132955=DIRECTION('center_axis',(-3.07718727278846E-18,-7.01224015889347E-15,
1.));
#132956=DIRECTION('ref_axis',(9.94952222982948E-36,-1.,-7.01224015889347E-15));
#132957=DIRECTION('center_axis',(-0.207911690817747,-0.978147600733808,
-6.85964567039976E-15));
#132958=DIRECTION('ref_axis',(3.07718727278847E-18,7.01224015889347E-15,
-1.));
#132959=DIRECTION('center_axis',(-0.207911690817745,-0.978147600733809,
-2.7567651637332E-15));
#132960=DIRECTION('ref_axis',(0.855538223402208,-0.181850263143641,0.484752338924096));
#132961=DIRECTION('',(-0.518344583061391,0.11017754233581,-0.848044693619241));
#132962=DIRECTION('',(0.978147600733808,-0.207911690817747,-1.45491676450776E-15));
#132963=DIRECTION('',(-0.518344070249268,0.110177433334218,0.848045021223111));
#132964=DIRECTION('center_axis',(-0.207911690817745,-0.978147600733809,
-7.09867191847369E-15));
#132965=DIRECTION('ref_axis',(0.855536389092356,-0.18184987324904,-0.484755722542933));
#132966=DIRECTION('',(-0.978147600733808,0.207911690817747,1.31409985761785E-15));
#132967=DIRECTION('',(-0.489078703542046,0.103956887610932,-0.866022509672745));
#132968=DIRECTION('center_axis',(0.207912616962018,0.978147403873933,-1.63998885026162E-6));
#132969=DIRECTION('ref_axis',(0.847146577451534,-0.180066563904072,0.499918702266611));
#132970=DIRECTION('',(-0.978147600733808,0.207911690817747,1.31409985761785E-15));
#132971=DIRECTION('center_axis',(0.207910764585284,0.978147797608763,-1.6401440529113E-6));
#132972=DIRECTION('ref_axis',(0.847118160921299,-0.18006052355587,-0.499969028334858));
#132973=DIRECTION('',(-0.489078856702219,0.103956920166105,0.86602241926894));
#132974=DIRECTION('',(-0.978147600733808,0.207911690817747,1.31409985761785E-15));
#132975=DIRECTION('center_axis',(-0.207911690817747,-0.978147600733808,
-6.85964567039976E-15));
#132976=DIRECTION('ref_axis',(3.07718727278847E-18,7.01224015889347E-15,
-1.));
#132977=DIRECTION('center_axis',(0.20791169081776,0.978147600733805,3.47352489950765E-14));
#132978=DIRECTION('ref_axis',(0.855536389075249,-0.181849873245405,-0.484755722574488));
#132979=DIRECTION('',(0.518344070249258,-0.110177433334215,-0.848045021223117));
#132980=DIRECTION('',(-0.978147600733808,0.207911690817747,1.45491676450776E-15));
#132981=DIRECTION('',(0.518344583061387,-0.110177542335809,0.848044693619244));
#132982=DIRECTION('center_axis',(0.207911690817735,0.978147600733811,2.13649300215755E-14));
#132983=DIRECTION('ref_axis',(0.855538223422491,-0.181850263147953,0.484752338886681));
#132984=DIRECTION('',(0.978147600733808,-0.207911690817747,-1.31409985761785E-15));
#132985=DIRECTION('',(0.489078856702207,-0.103956920166111,-0.866022419268947));
#132986=DIRECTION('center_axis',(-0.207912617177289,-0.978147403828175,
-1.64037042596789E-6));
#132987=DIRECTION('ref_axis',(0.847146677889706,-0.180066585253107,-0.499918524377443));
#132988=DIRECTION('',(0.978147600733808,-0.207911690817747,-1.31409985761785E-15));
#132989=DIRECTION('center_axis',(-0.207910764792045,-0.978147797564815,
-1.6397775832553E-6));
#132990=DIRECTION('ref_axis',(0.847118057040066,-0.180060501475481,0.499969212297179));
#132991=DIRECTION('',(0.489078703542049,-0.103956887610926,0.866022509672744));
#132992=DIRECTION('',(0.978147600733808,-0.207911690817747,-1.31409985761785E-15));
#132993=DIRECTION('center_axis',(-7.71409749858844E-19,-6.99768205256557E-15,
1.));
#132994=DIRECTION('ref_axis',(0.,-1.,-6.99768205256557E-15));
#132995=DIRECTION('',(0.994521895368275,-0.10452846326764,-7.3068976750369E-16));
#132996=DIRECTION('center_axis',(7.71409749858844E-19,6.99768205256557E-15,
-1.));
#132997=DIRECTION('ref_axis',(2.20623519453511E-12,-1.,-6.99768205256557E-15));
#132998=DIRECTION('',(-0.994521895368275,0.10452846326764,7.3068976750369E-16));
#132999=DIRECTION('center_axis',(-7.71409749858844E-19,-6.99768205256557E-15,
1.));
#133000=DIRECTION('ref_axis',(2.59899164973018E-36,-1.,-6.99768205256557E-15));
#133001=DIRECTION('center_axis',(-0.10452846326764,-0.994521895368275,-6.95942865237777E-15));
#133002=DIRECTION('ref_axis',(7.71409749858829E-19,6.99768205256557E-15,
-1.));
#133003=DIRECTION('center_axis',(-0.10452846326763,-0.994521895368276,-2.52933203772504E-14));
#133004=DIRECTION('ref_axis',(0.869860024050779,-0.0914259726160321,0.484752338921217));
#133005=DIRECTION('',(-0.527021726387077,0.0553922155203068,-0.848044693619232));
#133006=DIRECTION('',(0.994521895368275,-0.10452846326764,-7.3068976750369E-16));
#133007=DIRECTION('',(-0.527021204990414,0.0553921607192977,0.848045021223107));
#133008=DIRECTION('center_axis',(-0.104528463267641,-0.994521895368275,
-4.78988056634914E-15));
#133009=DIRECTION('ref_axis',(0.86985815903191,-0.091425776594645,-0.484755722544544));
#133010=DIRECTION('',(-0.994521895368275,0.10452846326764,5.89872860613779E-16));
#133011=DIRECTION('',(-0.497265932938972,0.0522647556052191,-0.866022509672734));
#133012=DIRECTION('center_axis',(0.104529404915855,0.994521796395256,-1.63998886015915E-6));
#133013=DIRECTION('ref_axis',(0.861327901070753,-0.0905292105226655,0.499918702269873));
#133014=DIRECTION('',(-0.994521895368275,0.10452846326764,5.89872860613779E-16));
#133015=DIRECTION('center_axis',(0.104527521530137,0.994521994347072,-1.64014407012473E-6));
#133016=DIRECTION('ref_axis',(0.8612990088216,-0.0905261736004439,-0.499969028336947));
#133017=DIRECTION('',(-0.497266088662992,0.0522647719724638,0.866022419268968));
#133018=DIRECTION('',(-0.994521895368275,0.10452846326764,5.89872860613779E-16));
#133019=DIRECTION('center_axis',(-0.10452846326764,-0.994521895368275,-6.95942865237777E-15));
#133020=DIRECTION('ref_axis',(7.71409749858829E-19,6.99768205256557E-15,
-1.));
#133021=DIRECTION('center_axis',(0.104528463267642,0.994521895368275,1.39905864007942E-14));
#133022=DIRECTION('ref_axis',(0.869858159014795,-0.0914257765928421,-0.484755722575595));
#133023=DIRECTION('',(0.527021204990409,-0.0553921607193002,-0.84804502122311));
#133024=DIRECTION('',(-0.994521895368275,0.10452846326764,7.3068976750369E-16));
#133025=DIRECTION('',(0.527021726387067,-0.0553922155203071,0.848044693619238));
#133026=DIRECTION('center_axis',(0.104528463267631,0.994521895368276,2.0158845262292E-14));
#133027=DIRECTION('ref_axis',(0.869860024068846,-0.0914259726179291,0.48475233888844));
#133028=DIRECTION('',(0.994521895368275,-0.10452846326764,-5.89872860613779E-16));
#133029=DIRECTION('',(0.497266088663057,-0.0522647719724677,-0.86602241926893));
#133030=DIRECTION('center_axis',(-0.104529405134737,-0.99452179637225,-1.64037044313809E-6));
#133031=DIRECTION('ref_axis',(0.861328003191411,-0.0905292212562206,-0.499918524378763));
#133032=DIRECTION('',(0.994521895368275,-0.10452846326764,-5.89872860613779E-16));
#133033=DIRECTION('center_axis',(-0.104527521740345,-0.994521994324979,
-1.63977763949909E-6));
#133034=DIRECTION('ref_axis',(0.861298903203584,-0.0905261624997945,0.499969212295481));
#133035=DIRECTION('',(0.497265932938949,-0.0522647556052211,0.866022509672747));
#133036=DIRECTION('',(0.994521895368275,-0.10452846326764,-5.89872860613779E-16));
#133037=DIRECTION('center_axis',(0.994521895368273,0.104528463267654,7.29146948004067E-16));
#133038=DIRECTION('ref_axis',(0.104528463267654,-0.994521895368273,-7.42349998278334E-15));
#133039=DIRECTION('center_axis',(-0.994521895368273,-0.104528463267654,
-7.29146948004067E-16));
#133040=DIRECTION('ref_axis',(-0.104528463267654,0.994521895368273,7.42349998278332E-15));
#133041=DIRECTION('center_axis',(0.978147600733806,0.20791169081776,1.44876238996227E-15));
#133042=DIRECTION('ref_axis',(0.20791169081776,-0.978147600733805,-7.42349998278335E-15));
#133043=DIRECTION('center_axis',(-0.978147600733806,-0.20791169081776,-1.44876238996227E-15));
#133044=DIRECTION('ref_axis',(-0.20791169081776,0.978147600733805,7.42349998278332E-15));
#133045=DIRECTION('center_axis',(0.951056516295153,0.309016994374948,2.15096206850332E-15));
#133046=DIRECTION('ref_axis',(0.309016994374948,-0.951056516295153,-7.42349998278335E-15));
#133047=DIRECTION('center_axis',(-0.951056516295153,-0.309016994374948,
-2.15096206850332E-15));
#133048=DIRECTION('ref_axis',(-0.309016994374948,0.951056516295153,7.42349998278333E-15));
#133049=DIRECTION('center_axis',(0.913545457642601,0.406736643075801,2.82805253700437E-15));
#133050=DIRECTION('ref_axis',(0.406736643075801,-0.913545457642601,-7.42349998278338E-15));
#133051=DIRECTION('center_axis',(-0.913545457642601,-0.406736643075801,
-2.82805253700437E-15));
#133052=DIRECTION('ref_axis',(-0.406736643075801,0.9135454576426,7.42349998278333E-15));
#133053=DIRECTION('center_axis',(0.866025403784438,0.500000000000001,3.47261545060224E-15));
#133054=DIRECTION('ref_axis',(0.500000000000001,-0.866025403784438,-4.94899998852227E-15));
#133055=DIRECTION('center_axis',(-0.866025403784438,-0.500000000000001,
-3.47261545060224E-15));
#133056=DIRECTION('ref_axis',(-0.500000000000001,0.866025403784438,4.94899998852221E-15));
#133057=DIRECTION('center_axis',(0.809016994374947,0.587785252292474,4.0775888431321E-15));
#133058=DIRECTION('ref_axis',(0.587785252292474,-0.809016994374947,-4.9489999885223E-15));
#133059=DIRECTION('center_axis',(-0.809016994374947,-0.587785252292474,
-4.0775888431321E-15));
#133060=DIRECTION('ref_axis',(-0.587785252292474,0.809016994374947,4.94899998852222E-15));
#133061=DIRECTION('center_axis',(0.743144825477393,0.669130606358859,4.63634449950655E-15));
#133062=DIRECTION('ref_axis',(0.669130606358859,-0.743144825477393,-4.94899998852211E-15));
#133063=DIRECTION('center_axis',(-0.743144825477393,-0.669130606358859,
-4.63634449950655E-15));
#133064=DIRECTION('ref_axis',(-0.669130606358859,0.743144825477393,4.94899998852222E-15));
#133065=DIRECTION('center_axis',(0.669130606358857,0.743144825477395,5.14276057582724E-15));
#133066=DIRECTION('ref_axis',(0.743144825477396,-0.669130606358857,-4.94899998852226E-15));
#133067=DIRECTION('center_axis',(-0.669130606358857,-0.743144825477395,
-5.14276057582724E-15));
#133068=DIRECTION('ref_axis',(-0.743144825477395,0.669130606358857,4.94899998852221E-15));
#133069=DIRECTION('center_axis',(0.587785252292471,0.809016994374949,5.59128867158761E-15));
#133070=DIRECTION('ref_axis',(0.809016994374949,-0.587785252292471,-4.94899998852211E-15));
#133071=DIRECTION('center_axis',(-0.587785252292471,-0.809016994374949,
-5.59128867158761E-15));
#133072=DIRECTION('ref_axis',(-0.809016994374949,0.587785252292472,4.94899998852222E-15));
#133073=DIRECTION('center_axis',(0.499999999999998,0.86602540378444,5.97701461910997E-15));
#133074=DIRECTION('ref_axis',(0.86602540378444,-0.499999999999998,-2.47449999426116E-15));
#133075=DIRECTION('center_axis',(-0.499999999999998,-0.86602540378444,-5.97701461910997E-15));
#133076=DIRECTION('ref_axis',(-0.86602540378444,0.499999999999998,2.47449999426111E-15));
#133077=DIRECTION('center_axis',(0.406736643075798,0.913545457642602,6.29571232419492E-15));
#133078=DIRECTION('ref_axis',(0.913545457642602,-0.406736643075798,-2.474499994261E-15));
#133079=DIRECTION('center_axis',(-0.406736643075798,-0.913545457642602,
-6.29571232419492E-15));
#133080=DIRECTION('ref_axis',(-0.913545457642602,0.406736643075798,2.47449999426111E-15));
#133081=DIRECTION('center_axis',(0.309016994374945,0.951056516295155,6.54389006809377E-15));
#133082=DIRECTION('ref_axis',(0.951056516295154,-0.309016994374945,-2.47449999426112E-15));
#133083=DIRECTION('center_axis',(-0.309016994374945,-0.951056516295155,
-6.54389006809377E-15));
#133084=DIRECTION('ref_axis',(-0.951056516295154,0.309016994374945,2.47449999426111E-15));
#133085=DIRECTION('center_axis',(0.207911690817756,0.978147600733806,6.71882876350984E-15));
#133086=DIRECTION('ref_axis',(0.978147600733806,-0.207911690817756,-2.47449999426122E-15));
#133087=DIRECTION('center_axis',(-0.207911690817756,-0.978147600733806,
-6.71882876350984E-15));
#133088=DIRECTION('ref_axis',(-0.978147600733806,0.207911690817756,2.47449999426111E-15));
#133089=DIRECTION('center_axis',(0.10452846326765,0.994521895368274,6.81861174548786E-15));
#133090=DIRECTION('ref_axis',(0.994521895368274,-0.10452846326765,-7.6256220630635E-29));
#133091=DIRECTION('center_axis',(-0.10452846326765,-0.994521895368274,-6.81861174548786E-15));
#133092=DIRECTION('ref_axis',(-0.994521895368274,0.10452846326765,5.35058014197221E-32));
#133093=DIRECTION('center_axis',(-3.49148133884313E-15,1.,6.84214577079636E-15));
#133094=DIRECTION('ref_axis',(1.,3.49148133884313E-15,2.38892242763799E-29));
#133095=DIRECTION('center_axis',(3.49148133884313E-15,-1.,-6.84214577079636E-15));
#133096=DIRECTION('ref_axis',(-1.,-3.49148133884313E-15,3.67140197653102E-43));
#133097=DIRECTION('center_axis',(-0.104528463267657,0.994521895368273,6.78917299572924E-15));
#133098=DIRECTION('ref_axis',(0.994521895368273,0.104528463267657,1.21818699066432E-28));
#133099=DIRECTION('center_axis',(0.104528463267657,-0.994521895368273,-6.78917299572924E-15));
#133100=DIRECTION('ref_axis',(-0.994521895368273,-0.104528463267657,-1.19282195192603E-32));
#133101=DIRECTION('center_axis',(-0.207911690817763,0.978147600733805,6.66027380109541E-15));
#133102=DIRECTION('ref_axis',(0.978147600733805,0.207911690817763,2.47449999426098E-15));
#133103=DIRECTION('center_axis',(0.207911690817763,-0.978147600733805,-6.66027380109541E-15));
#133104=DIRECTION('ref_axis',(-0.978147600733805,-0.207911690817763,-2.47449999426111E-15));
#133105=DIRECTION('center_axis',(-0.309016994374951,0.951056516295152,6.45686043344516E-15));
#133106=DIRECTION('ref_axis',(0.951056516295152,0.309016994374951,2.47449999426116E-15));
#133107=DIRECTION('center_axis',(0.309016994374951,-0.951056516295152,-6.45686043344516E-15));
#133108=DIRECTION('ref_axis',(-0.951056516295152,-0.309016994374951,-2.47449999426111E-15));
#133109=DIRECTION('center_axis',(-0.406736643075804,0.913545457642599,6.18116153220146E-15));
#133110=DIRECTION('ref_axis',(0.913545457642599,0.406736643075804,2.47449999426104E-15));
#133111=DIRECTION('center_axis',(0.406736643075804,-0.913545457642599,-6.18116153220146E-15));
#133112=DIRECTION('ref_axis',(-0.913545457642599,-0.406736643075804,-2.47449999426111E-15));
#133113=DIRECTION('center_axis',(-0.500000000000004,0.866025403784436,5.83619771222003E-15));
#133114=DIRECTION('ref_axis',(0.866025403784436,0.500000000000004,2.47449999426119E-15));
#133115=DIRECTION('center_axis',(0.500000000000004,-0.866025403784436,-5.83619771222003E-15));
#133116=DIRECTION('ref_axis',(-0.866025403784436,-0.500000000000004,-2.47449999426111E-15));
#133117=DIRECTION('center_axis',(-0.587785252292477,0.809016994374945,5.42574846930092E-15));
#133118=DIRECTION('ref_axis',(0.809016994374945,0.587785252292477,4.94899998852215E-15));
#133119=DIRECTION('center_axis',(0.587785252292477,-0.809016994374945,-5.42574846930092E-15));
#133120=DIRECTION('ref_axis',(-0.809016994374945,-0.587785252292477,-4.94899998852222E-15));
#133121=DIRECTION('center_axis',(-0.669130606358862,0.743144825477391,4.95431077124156E-15));
#133122=DIRECTION('ref_axis',(0.743144825477391,0.669130606358862,4.9489999885223E-15));
#133123=DIRECTION('center_axis',(0.669130606358862,-0.743144825477391,-4.95431077124156E-15));
#133124=DIRECTION('ref_axis',(-0.743144825477391,-0.669130606358862,-4.94899998852222E-15));
#133125=DIRECTION('center_axis',(-0.743144825477398,0.669130606358854,4.42704978811658E-15));
#133126=DIRECTION('ref_axis',(0.669130606358854,0.743144825477398,4.94899998852214E-15));
#133127=DIRECTION('center_axis',(0.743144825477398,-0.669130606358854,-4.42704978811658E-15));
#133128=DIRECTION('ref_axis',(-0.669130606358854,-0.743144825477398,-4.94899998852222E-15));
#133129=DIRECTION('center_axis',(-0.809016994374951,0.587785252292469,3.84974230159355E-15));
#133130=DIRECTION('ref_axis',(0.587785252292469,0.80901699437495,4.94899998852232E-15));
#133131=DIRECTION('center_axis',(0.809016994374951,-0.587785252292469,-3.84974230159355E-15));
#133132=DIRECTION('ref_axis',(-0.587785252292469,-0.809016994374951,-4.94899998852222E-15));
#133133=DIRECTION('center_axis',(-0.866025403784442,0.499999999999995,3.22871341330418E-15));
#133134=DIRECTION('ref_axis',(0.499999999999995,0.866025403784442,4.94899998852218E-15));
#133135=DIRECTION('center_axis',(0.866025403784442,-0.499999999999995,-3.22871341330418E-15));
#133136=DIRECTION('ref_axis',(-0.499999999999995,-0.866025403784442,-4.94899998852222E-15));
#133137=DIRECTION('center_axis',(-0.913545457642603,0.406736643075795,2.57076724570721E-15));
#133138=DIRECTION('ref_axis',(0.406736643075795,0.913545457642603,7.42349998278324E-15));
#133139=DIRECTION('center_axis',(0.913545457642603,-0.406736643075795,-2.57076724570721E-15));
#133140=DIRECTION('ref_axis',(-0.406736643075795,-0.913545457642603,-7.42349998278332E-15));
#133141=DIRECTION('center_axis',(-0.951056516295156,0.309016994374942,1.88311239469892E-15));
#133142=DIRECTION('ref_axis',(0.309016994374942,0.951056516295155,7.42349998278336E-15));
#133143=DIRECTION('center_axis',(0.951056516295156,-0.309016994374942,-1.88311239469892E-15));
#133144=DIRECTION('ref_axis',(-0.309016994374942,-0.951056516295156,-7.42349998278332E-15));
#133145=DIRECTION('center_axis',(-0.978147600733807,0.207911690817753,1.17328295072799E-15));
#133146=DIRECTION('ref_axis',(0.207911690817753,0.978147600733807,7.42349998278336E-15));
#133147=DIRECTION('center_axis',(0.978147600733807,-0.207911690817753,-1.17328295072799E-15));
#133148=DIRECTION('ref_axis',(-0.207911690817753,-0.978147600733807,-7.42349998278332E-15));
#133149=DIRECTION('center_axis',(-0.994521895368274,0.104528463267647,4.49055953723918E-16));
#133150=DIRECTION('ref_axis',(0.104528463267647,0.994521895368274,7.42349998278331E-15));
#133151=DIRECTION('center_axis',(0.994521895368274,-0.104528463267647,-4.49055953723918E-16));
#133152=DIRECTION('ref_axis',(-0.104528463267647,-0.994521895368274,-7.42349998278332E-15));
#133153=DIRECTION('center_axis',(-1.,1.96663841039893E-30,-2.81633813779821E-16));
#133154=DIRECTION('ref_axis',(2.81633813779821E-16,6.97886326506453E-15,
-1.));
#133155=DIRECTION('center_axis',(1.,-1.96663841039893E-30,2.81633813779821E-16));
#133156=DIRECTION('ref_axis',(-2.81633813779821E-16,-6.97886326506453E-15,
1.));
#133157=DIRECTION('center_axis',(-0.994521895368273,-0.104528463267661,
-1.01078076178394E-15));
#133158=DIRECTION('ref_axis',(-0.104528463267661,0.994521895368273,7.42349998278334E-15));
#133159=DIRECTION('center_axis',(0.994521895368273,0.104528463267661,1.01078076178394E-15));
#133160=DIRECTION('ref_axis',(0.104528463267661,-0.994521895368273,-7.42349998278332E-15));
#133161=DIRECTION('center_axis',(-0.978147600733804,-0.207911690817766,
-1.73039620374214E-15));
#133162=DIRECTION('ref_axis',(-0.207911690817766,0.978147600733804,7.42349998278333E-15));
#133163=DIRECTION('center_axis',(0.978147600733804,0.207911690817766,1.73039620374214E-15));
#133164=DIRECTION('ref_axis',(0.207911690817766,-0.978147600733804,-7.42349998278332E-15));
#133165=DIRECTION('center_axis',(-0.951056516295151,-0.309016994374955,
-2.43259588228318E-15));
#133166=DIRECTION('ref_axis',(-0.309016994374955,0.951056516295151,7.42349998278333E-15));
#133167=DIRECTION('center_axis',(0.951056516295151,0.309016994374955,2.43259588228318E-15));
#133168=DIRECTION('ref_axis',(0.309016994374954,-0.951056516295151,-7.42349998278332E-15));
#133169=DIRECTION('center_axis',(-0.913545457642598,-0.406736643075807,
-3.10968635078423E-15));
#133170=DIRECTION('ref_axis',(-0.406736643075807,0.913545457642598,7.42349998278337E-15));
#133171=DIRECTION('center_axis',(0.913545457642598,0.406736643075807,3.10968635078423E-15));
#133172=DIRECTION('ref_axis',(0.406736643075807,-0.913545457642598,-7.42349998278332E-15));
#133173=DIRECTION('center_axis',(-0.866025403784435,-0.500000000000007,
-3.7542492643821E-15));
#133174=DIRECTION('ref_axis',(-0.500000000000007,0.866025403784435,4.94899998852224E-15));
#133175=DIRECTION('center_axis',(0.866025403784435,0.500000000000007,3.7542492643821E-15));
#133176=DIRECTION('ref_axis',(0.500000000000007,-0.866025403784435,-4.94899998852222E-15));
#133177=DIRECTION('center_axis',(-0.809016994374943,-0.58778525229248,-4.35922265691196E-15));
#133178=DIRECTION('ref_axis',(-0.58778525229248,0.809016994374943,4.94899998852228E-15));
#133179=DIRECTION('center_axis',(0.809016994374943,0.58778525229248,4.35922265691196E-15));
#133180=DIRECTION('ref_axis',(0.58778525229248,-0.809016994374943,-4.94899998852221E-15));
#133181=DIRECTION('center_axis',(-0.743144825477389,-0.669130606358864,
-4.91797831328641E-15));
#133182=DIRECTION('ref_axis',(-0.669130606358864,0.743144825477389,4.94899998852235E-15));
#133183=DIRECTION('center_axis',(0.743144825477389,0.669130606358864,4.91797831328641E-15));
#133184=DIRECTION('ref_axis',(0.669130606358864,-0.743144825477388,-4.94899998852221E-15));
#133185=DIRECTION('center_axis',(-0.669130606358852,-0.7431448254774,-5.42439438960709E-15));
#133186=DIRECTION('ref_axis',(-0.7431448254774,0.669130606358852,4.94899998852223E-15));
#133187=DIRECTION('center_axis',(0.669130606358852,0.7431448254774,5.42439438960709E-15));
#133188=DIRECTION('ref_axis',(0.7431448254774,-0.669130606358852,-4.94899998852222E-15));
#133189=DIRECTION('center_axis',(-0.587785252292466,-0.809016994374953,
-5.87292248536745E-15));
#133190=DIRECTION('ref_axis',(-0.809016994374953,0.587785252292466,4.94899998852237E-15));
#133191=DIRECTION('center_axis',(0.587785252292466,0.809016994374953,5.87292248536745E-15));
#133192=DIRECTION('ref_axis',(0.809016994374953,-0.587785252292466,-4.94899998852222E-15));
#133193=DIRECTION('center_axis',(-0.499999999999992,-0.866025403784443,
-6.25864843288981E-15));
#133194=DIRECTION('ref_axis',(-0.866025403784443,0.499999999999992,2.47449999426112E-15));
#133195=DIRECTION('center_axis',(0.499999999999992,0.866025403784443,6.25864843288981E-15));
#133196=DIRECTION('ref_axis',(0.866025403784443,-0.499999999999992,-2.47449999426111E-15));
#133197=DIRECTION('center_axis',(-0.406736643075792,-0.913545457642605,
-6.57734613797476E-15));
#133198=DIRECTION('ref_axis',(-0.913545457642605,0.406736643075792,2.47449999426124E-15));
#133199=DIRECTION('center_axis',(0.406736643075792,0.913545457642605,6.57734613797476E-15));
#133200=DIRECTION('ref_axis',(0.913545457642605,-0.406736643075792,-2.47449999426111E-15));
#133201=DIRECTION('center_axis',(-0.309016994374938,-0.951056516295157,
-6.82552388187361E-15));
#133202=DIRECTION('ref_axis',(-0.951056516295157,0.309016994374938,2.47449999426107E-15));
#133203=DIRECTION('center_axis',(0.309016994374938,0.951056516295157,6.82552388187361E-15));
#133204=DIRECTION('ref_axis',(0.951056516295157,-0.309016994374938,-2.47449999426111E-15));
#133205=DIRECTION('center_axis',(-0.207911690817749,-0.978147600733808,
-7.00046257728967E-15));
#133206=DIRECTION('ref_axis',(-0.978147600733808,0.207911690817749,2.47449999426117E-15));
#133207=DIRECTION('center_axis',(0.207911690817749,0.978147600733808,7.00046257728967E-15));
#133208=DIRECTION('ref_axis',(0.978147600733808,-0.207911690817749,-2.47449999426111E-15));
#133209=DIRECTION('center_axis',(-0.104528463267644,-0.994521895368275,
-7.10024555926768E-15));
#133210=DIRECTION('ref_axis',(-0.994521895368274,0.104528463267644,3.50875041575624E-29));
#133211=DIRECTION('center_axis',(0.104528463267644,0.994521895368275,7.10024555926768E-15));
#133212=DIRECTION('ref_axis',(0.994521895368274,-0.104528463267644,-7.58109811812969E-32));
#133213=DIRECTION('center_axis',(1.04744440165294E-14,-1.,-7.12377958457618E-15));
#133214=DIRECTION('ref_axis',(-1.,-1.04744440165294E-14,-7.46176304447382E-29));
#133215=DIRECTION('center_axis',(-1.04744440165294E-14,1.,7.12377958457618E-15));
#133216=DIRECTION('ref_axis',(1.,1.04744440165294E-14,-1.5694542800438E-43));
#133217=DIRECTION('center_axis',(0.104528463267664,-0.994521895368272,-7.07080680950905E-15));
#133218=DIRECTION('ref_axis',(-0.994521895368272,-0.104528463267664,1.05361876330055E-28));
#133219=DIRECTION('center_axis',(-0.104528463267664,0.994521895368272,7.07080680950905E-15));
#133220=DIRECTION('ref_axis',(0.994521895368272,0.104528463267664,-1.29041391784167E-31));
#133221=DIRECTION('center_axis',(0.20791169081777,-0.978147600733803,-6.94190761487522E-15));
#133222=DIRECTION('ref_axis',(-0.978147600733803,-0.20791169081777,-2.47449999426102E-15));
#133223=DIRECTION('center_axis',(-0.20791169081777,0.978147600733803,6.94190761487522E-15));
#133224=DIRECTION('ref_axis',(0.978147600733803,0.20791169081777,2.47449999426111E-15));
#133225=DIRECTION('center_axis',(0.309016994374957,-0.95105651629515,-6.73849424722497E-15));
#133226=DIRECTION('ref_axis',(-0.95105651629515,-0.309016994374957,-2.47449999426121E-15));
#133227=DIRECTION('center_axis',(-0.309016994374957,0.95105651629515,6.73849424722497E-15));
#133228=DIRECTION('ref_axis',(0.95105651629515,0.309016994374957,2.47449999426111E-15));
#133229=DIRECTION('center_axis',(0.40673664307581,-0.913545457642596,-6.46279534598126E-15));
#133230=DIRECTION('ref_axis',(-0.913545457642597,-0.40673664307581,-2.47449999426108E-15));
#133231=DIRECTION('center_axis',(-0.40673664307581,0.913545457642596,6.46279534598126E-15));
#133232=DIRECTION('ref_axis',(0.913545457642596,0.40673664307581,2.47449999426111E-15));
#133233=DIRECTION('center_axis',(0.50000000000001,-0.866025403784433,-6.11783152599983E-15));
#133234=DIRECTION('ref_axis',(-0.866025403784433,-0.50000000000001,-2.47449999426098E-15));
#133235=DIRECTION('center_axis',(-0.50000000000001,0.866025403784433,6.11783152599983E-15));
#133236=DIRECTION('ref_axis',(0.866025403784433,0.50000000000001,2.47449999426111E-15));
#133237=DIRECTION('center_axis',(0.587785252292482,-0.809016994374941,-5.70738228308071E-15));
#133238=DIRECTION('ref_axis',(-0.809016994374941,-0.587785252292482,-4.94899998852218E-15));
#133239=DIRECTION('center_axis',(-0.587785252292482,0.809016994374941,5.70738228308071E-15));
#133240=DIRECTION('ref_axis',(0.809016994374941,0.587785252292482,4.94899998852221E-15));
#133241=DIRECTION('center_axis',(0.669130606358867,-0.743144825477386,-5.23594458502135E-15));
#133242=DIRECTION('ref_axis',(-0.743144825477386,-0.669130606358867,-4.94899998852234E-15));
#133243=DIRECTION('center_axis',(-0.669130606358867,0.743144825477386,5.23594458502135E-15));
#133244=DIRECTION('ref_axis',(0.743144825477386,0.669130606358867,4.94899998852222E-15));
#133245=DIRECTION('center_axis',(0.743144825477402,-0.66913060635885,-4.70868360189637E-15));
#133246=DIRECTION('ref_axis',(-0.66913060635885,-0.743144825477402,-4.94899998852217E-15));
#133247=DIRECTION('center_axis',(-0.743144825477402,0.66913060635885,4.70868360189637E-15));
#133248=DIRECTION('ref_axis',(0.66913060635885,0.743144825477402,4.94899998852222E-15));
#133249=DIRECTION('center_axis',(0.809016994374955,-0.587785252292463,-4.13137611537334E-15));
#133250=DIRECTION('ref_axis',(-0.587785252292463,-0.809016994374955,-4.94899998852209E-15));
#133251=DIRECTION('center_axis',(-0.809016994374955,0.587785252292463,4.13137611537334E-15));
#133252=DIRECTION('ref_axis',(0.587785252292463,0.809016994374955,4.94899998852222E-15));
#133253=DIRECTION('center_axis',(0.866025403784445,-0.499999999999989,-3.51034722708396E-15));
#133254=DIRECTION('ref_axis',(-0.499999999999989,-0.866025403784445,-4.9489999885222E-15));
#133255=DIRECTION('center_axis',(-0.866025403784445,0.499999999999989,3.51034722708396E-15));
#133256=DIRECTION('ref_axis',(0.499999999999989,0.866025403784445,4.94899998852222E-15));
#133257=DIRECTION('center_axis',(0.913545457642606,-0.406736643075789,-2.85240105948698E-15));
#133258=DIRECTION('ref_axis',(-0.406736643075789,-0.913545457642606,-7.42349998278328E-15));
#133259=DIRECTION('center_axis',(-0.913545457642606,0.406736643075789,2.85240105948698E-15));
#133260=DIRECTION('ref_axis',(0.406736643075789,0.913545457642606,7.42349998278333E-15));
#133261=DIRECTION('center_axis',(0.951056516295158,-0.309016994374935,-2.16474620847869E-15));
#133262=DIRECTION('ref_axis',(-0.309016994374935,-0.951056516295158,-7.42349998278338E-15));
#133263=DIRECTION('center_axis',(-0.951056516295158,0.309016994374935,2.16474620847869E-15));
#133264=DIRECTION('ref_axis',(0.309016994374935,0.951056516295158,7.42349998278332E-15));
#133265=DIRECTION('center_axis',(0.978147600733808,-0.207911690817747,-1.45491676450776E-15));
#133266=DIRECTION('ref_axis',(-0.207911690817747,-0.978147600733808,-7.42349998278336E-15));
#133267=DIRECTION('center_axis',(-0.978147600733808,0.207911690817747,1.45491676450776E-15));
#133268=DIRECTION('ref_axis',(0.207911690817747,0.978147600733808,7.42349998278332E-15));
#133269=DIRECTION('center_axis',(0.994521895368275,-0.10452846326764,-7.3068976750369E-16));
#133270=DIRECTION('ref_axis',(-0.10452846326764,-0.994521895368275,-7.42349998278331E-15));
#133271=DIRECTION('center_axis',(-0.994521895368275,0.10452846326764,7.3068976750369E-16));
#133272=DIRECTION('ref_axis',(0.10452846326764,0.994521895368275,7.42349998278333E-15));
#133273=DIRECTION('center_axis',(-0.497265934576059,-0.0522647557772786,
-0.866022508722343));
#133274=DIRECTION('ref_axis',(0.104528463272604,-0.994521895367753,-2.8717186175955E-12));
#133275=DIRECTION('center_axis',(-0.861277224843021,-0.0904936763726118,
-0.500012436348611));
#133276=DIRECTION('ref_axis',(0.49716964624235,0.0532497882929787,-0.866017784402843));
#133277=DIRECTION('center_axis',(0.497265943181924,0.0522647566817827,0.866022503726309));
#133278=DIRECTION('ref_axis',(-0.867207748104374,-7.42381499369421E-15,
0.497946504785143));
#133279=DIRECTION('center_axis',(0.994521895368276,0.104528463267628,7.29918357753749E-16));
#133280=DIRECTION('ref_axis',(0.104528463267628,-0.994521895368276,-6.82961998416064E-15));
#133281=DIRECTION('center_axis',(-0.994521895368273,-0.104528463267654,
-8.69963854893977E-16));
#133282=DIRECTION('ref_axis',(-0.104528463267654,0.994521895368273,6.82961998416066E-15));
#133283=DIRECTION('center_axis',(-0.994521895368276,-0.104528463267629,
6.97861005538628E-16));
#133284=DIRECTION('ref_axis',(-0.104528463267629,0.994521895368276,6.82961998416064E-15));
#133285=DIRECTION('center_axis',(-0.994521895368273,-0.104528463267654,
-8.69963854893977E-16));
#133286=DIRECTION('ref_axis',(-0.104528463267654,0.994521895368273,6.82961998416066E-15));
#133287=DIRECTION('center_axis',(0.994521895368276,0.104528463267628,7.29918357753744E-16));
#133288=DIRECTION('ref_axis',(0.104528463267628,-0.994521895368276,-6.82961998416064E-15));
#133289=DIRECTION('center_axis',(-0.527021232978597,-0.0553921636609822,
0.848045003637587));
#133290=DIRECTION('ref_axis',(-0.849349030019387,7.20117432794764E-15,-0.527831625809903));
#133291=DIRECTION('center_axis',(0.497266077958583,0.0522647708474123,-0.866022425483287));
#133292=DIRECTION('ref_axis',(0.867207670398076,-6.88055504554487E-15,0.497946640115929));
#133293=DIRECTION('center_axis',(0.527021202611631,0.055392182212892,-0.848045021297504));
#133294=DIRECTION('ref_axis',(0.842941044395307,0.0929299148191017,0.529919264233208));
#133295=DIRECTION('center_axis',(-0.527021177161361,-0.0553921577943543,
0.84804503870864));
#133296=DIRECTION('ref_axis',(-0.84934906486751,6.64538535710706E-15,-0.527831569734783));
#133297=DIRECTION('center_axis',(0.497266090635357,0.0522647827543777,-0.866022417485752));
#133298=DIRECTION('ref_axis',(0.860793892490753,0.0950466972103146,0.500000000000028));
#133299=DIRECTION('center_axis',(0.861296695145007,0.0904912830031523,-0.499979330205491));
#133300=DIRECTION('ref_axis',(0.49734089486934,0.0513033470000485,0.866036951219264));
#133301=DIRECTION('center_axis',(-0.104769627595161,0.994496518411991,1.52498774835248E-16));
#133302=DIRECTION('ref_axis',(0.994496518411991,0.104769627595161,7.18497231411654E-31));
#133303=DIRECTION('center_axis',(-0.994521895368273,-0.104528463267654,
-8.69963854893977E-16));
#133304=DIRECTION('ref_axis',(-0.104528463267654,0.994521895368273,6.82961998416066E-15));
#133305=DIRECTION('center_axis',(0.994521895368276,0.104528463267627,7.29918357753739E-16));
#133306=DIRECTION('ref_axis',(0.104528463267627,-0.994521895368276,-6.82961998416064E-15));
#133307=DIRECTION('center_axis',(-7.71409749859041E-19,-6.96824330280696E-15,
1.));
#133308=DIRECTION('ref_axis',(0.,-1.,-6.96738351343764E-15));
#133309=DIRECTION('center_axis',(-0.104287292793436,0.994547213842468,6.94488607545882E-15));
#133310=DIRECTION('ref_axis',(0.994547213842468,0.104287292793436,3.36172022659011E-29));
#133311=DIRECTION('center_axis',(0.52702169399903,0.0553922121162167,0.848044713969296));
#133312=DIRECTION('ref_axis',(-0.849348742192381,-6.70998093352327E-15,
0.527832088960325));
#133313=DIRECTION('center_axis',(0.52702117716142,0.055392157794407,-0.8480450387086));
#133314=DIRECTION('ref_axis',(0.849349064867473,-6.23548807247744E-15,0.527831569734843));
#133315=DIRECTION('center_axis',(0.52702172906978,0.0553921904544422,0.848044693589293));
#133316=DIRECTION('ref_axis',(-0.842916495802168,-0.0931523188070211,0.529919264233212));
#133317=DIRECTION('center_axis',(0.527021758969982,0.0553922189448927,0.848044673146732));
#133318=DIRECTION('ref_axis',(-0.849348701629304,-6.73646265345537E-15,
0.527832154231452));
#133319=DIRECTION('center_axis',(-0.527021202762452,-0.0553921822924323,
0.84804502119858));
#133320=DIRECTION('ref_axis',(0.843841975851294,0.0843581245990787,0.529919264233252));
#133321=DIRECTION('center_axis',(0.527021232978612,0.0553921636609838,-0.848045003637577));
#133322=DIRECTION('ref_axis',(0.849349030019378,-7.37535688457201E-15,0.527831625809918));
#133323=DIRECTION('center_axis',(-0.10478522557409,0.994494875050338,6.94452059562678E-15));
#133324=DIRECTION('ref_axis',(0.994494875050338,0.10478522557409,-6.10576890204024E-30));
#133325=DIRECTION('center_axis',(0.994521895368276,0.104528463267629,7.29918357753754E-16));
#133326=DIRECTION('ref_axis',(0.104528463267629,-0.994521895368276,-6.82961998416064E-15));
#133327=DIRECTION('center_axis',(-7.71409749859041E-19,-6.96824330280696E-15,
1.));
#133328=DIRECTION('ref_axis',(0.,-1.,-6.96662863860695E-15));
#133329=DIRECTION('center_axis',(-0.104271693993672,0.994548849394382,1.52506799409043E-16));
#133330=DIRECTION('ref_axis',(0.994548849394382,0.104271693993672,4.10784825130666E-32));
#133331=DIRECTION('center_axis',(0.994521895368273,0.104528463267654,8.69963854893977E-16));
#133332=DIRECTION('ref_axis',(0.104528463267654,-0.994521895368273,-6.82961998416066E-15));
#133333=DIRECTION('center_axis',(0.861270944310205,0.0905534316534015,0.500012436348137));
#133334=DIRECTION('ref_axis',(0.497376550147764,0.0512812291253674,-0.866017784403127));
#133335=DIRECTION('center_axis',(-0.527021758969975,-0.0553922189448919,
-0.848044673146736));
#133336=DIRECTION('ref_axis',(0.849348701629309,6.90235289882492E-15,-0.527832154231445));
#133337=DIRECTION('center_axis',(-0.497265930898087,-0.0522647452161537,
-0.866022511471584));
#133338=DIRECTION('ref_axis',(-0.861737632556767,-0.0860712067739632,0.499999999999932));
#133339=DIRECTION('center_axis',(0.497265943181814,0.0522647566817715,0.866022503726373));
#133340=DIRECTION('ref_axis',(-0.867207748104437,-6.28489530937578E-15,
0.497946504785033));
#133341=DIRECTION('center_axis',(-0.527021728885167,-0.0553921903536622,
-0.848044693710605));
#133342=DIRECTION('ref_axis',(-0.843864204094708,-0.0841354767153469,0.529919264233228));
#133343=DIRECTION('center_axis',(-0.527021693998979,-0.0553922121161939,
-0.848044713969329));
#133344=DIRECTION('ref_axis',(0.849348742192414,5.97509586698296E-15,-0.527832088960272));
#133345=DIRECTION('center_axis',(0.994521895368276,0.104528463267629,7.29918357753754E-16));
#133346=DIRECTION('ref_axis',(0.104528463267629,-0.994521895368276,-6.82961998416064E-15));
#133347=DIRECTION('center_axis',(-0.994521895368276,-0.104528463267629,
-7.29918357753754E-16));
#133348=DIRECTION('ref_axis',(-0.104528463267629,0.994521895368276,6.82961998416064E-15));
#133349=DIRECTION('center_axis',(0.994521895368273,0.104528463267654,8.69963854893977E-16));
#133350=DIRECTION('ref_axis',(0.104528463267654,-0.994521895368273,-6.82961998416066E-15));
#133351=DIRECTION('center_axis',(0.994521895368276,0.104528463267629,1.44380803939994E-15));
#133352=DIRECTION('ref_axis',(0.104528463267629,-0.994521895368276,-6.82961998416064E-15));
#133353=DIRECTION('center_axis',(0.994521895368273,0.104528463267654,8.69963854893977E-16));
#133354=DIRECTION('ref_axis',(0.104528463267654,-0.994521895368273,-6.82961998416066E-15));
#133355=DIRECTION('center_axis',(-0.861289491529676,-0.0905598208268648,
0.499979330205117));
#133356=DIRECTION('ref_axis',(0.497139368682041,0.0532207405894839,0.866036951219478));
#133357=DIRECTION('center_axis',(0.497266077958573,0.0522647708473918,-0.866022425483294));
#133358=DIRECTION('ref_axis',(0.867207670398082,-6.72680058735007E-15,0.497946640115918));
#133359=DIRECTION('center_axis',(0.497266086881507,0.0522647717852377,-0.866022420303188));
#133360=DIRECTION('ref_axis',(-0.104528463263061,0.994521895368756,2.66191267869619E-12));
#133361=DIRECTION('center_axis',(-0.489078705153339,-0.103956887953411,
-0.86602250872167));
#133362=DIRECTION('ref_axis',(0.207911690816915,-0.978147600733985,4.76434291194686E-13));
#133363=DIRECTION('center_axis',(-0.847099893161541,-0.18002592730432,-0.500012436349263));
#133364=DIRECTION('ref_axis',(0.488879980353917,0.104926459522144,-0.866017784402435));
#133365=DIRECTION('center_axis',(0.489078713616375,0.103956889752287,0.866022503726308));
#133366=DIRECTION('ref_axis',(-0.8707403454847,2.60936961613722E-16,0.491743073916842));
#133367=DIRECTION('center_axis',(0.978147600733807,0.207911690817754,1.45183957723502E-15));
#133368=DIRECTION('ref_axis',(0.207911690817754,-0.978147600733807,-6.8296199841607E-15));
#133369=DIRECTION('center_axis',(-0.978147600733806,-0.20791169081776,-1.58957929685218E-15));
#133370=DIRECTION('ref_axis',(-0.20791169081776,0.978147600733805,6.82961998416066E-15));
#133371=DIRECTION('center_axis',(-0.978147600733806,-0.207911690817757,
-1.45183957723504E-15));
#133372=DIRECTION('ref_axis',(-0.207911690817757,0.978147600733806,6.8296199841607E-15));
#133373=DIRECTION('center_axis',(-0.978147600733806,-0.20791169081776,-1.58957929685218E-15));
#133374=DIRECTION('ref_axis',(-0.20791169081776,0.978147600733805,6.82961998416066E-15));
#133375=DIRECTION('center_axis',(0.978147600733806,0.207911690817757,1.45183957723504E-15));
#133376=DIRECTION('ref_axis',(0.207911690817757,-0.978147600733806,-6.8296199841607E-15));
#133377=DIRECTION('center_axis',(-0.518344097776643,-0.110177439185358,
0.848045003637587));
#133378=DIRECTION('ref_axis',(-0.853239582811875,1.09365286413532E-15,-0.521519140898029));
#133379=DIRECTION('center_axis',(0.489078846174041,0.103956917928299,-0.866022425483266));
#133380=DIRECTION('ref_axis',(0.870740269393754,-1.06873346547645E-15,0.491743208652741));
#133381=DIRECTION('center_axis',(0.518344065636772,0.110177454461713,-0.848045021297501));
#133382=DIRECTION('ref_axis',(0.828609503968484,0.180532167016336,0.529919264233232));
#133383=DIRECTION('center_axis',(-0.518344042878402,-0.110177427516376,
0.848045038708645));
#133384=DIRECTION('ref_axis',(-0.853239616987301,5.33563410317125E-16,-0.521519084984782));
#133385=DIRECTION('center_axis',(0.489078857536798,0.103956931094697,-0.866022417485756));
#133386=DIRECTION('ref_axis',(0.846143288283833,0.18450348422784,0.50000000000001));
#133387=DIRECTION('center_axis',(0.847119506978957,0.180025582247261,-0.499979330205024));
#133388=DIRECTION('ref_axis',(0.489253749387828,0.10300858135289,0.86603695121953));
#133389=DIRECTION('center_axis',(-0.208148881407599,0.978097154258597,6.83001592333893E-15));
#133390=DIRECTION('ref_axis',(0.978097154258597,0.2081488814076,6.48647463947594E-29));
#133391=DIRECTION('center_axis',(-0.978147600733806,-0.20791169081776,-1.58957929685218E-15));
#133392=DIRECTION('ref_axis',(-0.20791169081776,0.978147600733805,6.82961998416066E-15));
#133393=DIRECTION('center_axis',(0.978147600733806,0.207911690817757,1.45183957723504E-15));
#133394=DIRECTION('ref_axis',(0.207911690817757,-0.978147600733806,-6.8296199841607E-15));
#133395=DIRECTION('center_axis',(-3.07718727278886E-18,-6.95368519647906E-15,
1.));
#133396=DIRECTION('ref_axis',(0.,-1.,-6.95327949822825E-15));
#133397=DIRECTION('center_axis',(-0.20767448800182,0.978197989689808,6.83072005339167E-15));
#133398=DIRECTION('ref_axis',(0.978197989689808,0.20767448800182,-2.3436552753213E-29));
#133399=DIRECTION('center_axis',(0.518344551206617,0.110177535564844,0.848044713969298));
#133400=DIRECTION('ref_axis',(-0.85323930054102,1.72522091353502E-16,0.521519602711414));
#133401=DIRECTION('center_axis',(0.518344042878406,0.110177427516377,-0.848045038708642));
#133402=DIRECTION('ref_axis',(0.853239616987298,-7.31872120548215E-16,0.521519084984786));
#133403=DIRECTION('center_axis',(0.518344588350353,0.110177517683876,0.848044693589272));
#133404=DIRECTION('ref_axis',(-0.828561842307896,-0.18075078662581,0.529919264233238));
#133405=DIRECTION('center_axis',(0.518344615107834,0.110177549147485,0.848044673146742));
#133406=DIRECTION('ref_axis',(-0.853239260760976,1.17359536946331E-15,0.521519667794095));
#133407=DIRECTION('center_axis',(-0.518344065777961,-0.11017745455898,0.848045021198566));
#133408=DIRECTION('ref_axis',(0.830401496091911,0.172101506916234,0.52991926423322));
#133409=DIRECTION('center_axis',(0.518344097776693,0.110177439185368,-0.848045003637555));
#133410=DIRECTION('ref_axis',(0.853239582811844,2.59696859442649E-16,0.52151914089808));
#133411=DIRECTION('center_axis',(-0.208164222161104,0.978093889466682,6.82999312541884E-15));
#133412=DIRECTION('ref_axis',(0.978093889466682,0.208164222161104,3.86600523032468E-29));
#133413=DIRECTION('center_axis',(0.978147600733806,0.207911690817757,1.45183957723504E-15));
#133414=DIRECTION('ref_axis',(0.207911690817757,-0.978147600733806,-6.8296199841607E-15));
#133415=DIRECTION('center_axis',(-3.07718727278886E-18,-6.95368519647906E-15,
1.));
#133416=DIRECTION('ref_axis',(0.,-1.,-6.95161435274788E-15));
#133417=DIRECTION('center_axis',(-0.207659145615656,0.978201246800563,6.8307427976745E-15));
#133418=DIRECTION('ref_axis',(0.978201246800563,0.207659145615656,5.37895539563461E-29));
#133419=DIRECTION('center_axis',(0.978147600733806,0.20791169081776,1.58957929685218E-15));
#133420=DIRECTION('ref_axis',(0.20791169081776,-0.978147600733806,-6.82961998416069E-15));
#133421=DIRECTION('center_axis',(0.847087400906439,0.18008469874752,0.500012436347927));
#133422=DIRECTION('ref_axis',(0.489291521298834,0.102990311594979,-0.866017784403208));
#133423=DIRECTION('center_axis',(-0.518344615107832,-0.110177549147514,
-0.84804467314674));
#133424=DIRECTION('ref_axis',(0.853239260760976,-1.16622482208424E-15,-0.521519667794095));
#133425=DIRECTION('center_axis',(-0.489078702596298,-0.103956877075459,
-0.866022511471521));
#133426=DIRECTION('ref_axis',(-0.84802005266229,-0.175675810180602,0.500000000000036));
#133427=DIRECTION('center_axis',(0.489078713616259,0.103956889752262,0.866022503726376));
#133428=DIRECTION('ref_axis',(-0.870740345484766,-4.19511635357395E-16,
0.491743073916725));
#133429=DIRECTION('center_axis',(-0.518344588177165,-0.110177517564694,
-0.848044693710613));
#133430=DIRECTION('ref_axis',(-0.830446875605574,-0.171882402215915,0.529919264233172));
#133431=DIRECTION('center_axis',(-0.518344551206558,-0.110177535564878,
-0.84804471396933));
#133432=DIRECTION('ref_axis',(0.853239300541055,-1.32448832729202E-15,-0.521519602711356));
#133433=DIRECTION('center_axis',(0.978147600733806,0.207911690817757,1.45183957723504E-15));
#133434=DIRECTION('ref_axis',(0.207911690817757,-0.978147600733806,-6.8296199841607E-15));
#133435=DIRECTION('center_axis',(-0.978147600733806,-0.207911690817757,
-1.45183957723504E-15));
#133436=DIRECTION('ref_axis',(-0.207911690817757,0.978147600733806,6.8296199841607E-15));
#133437=DIRECTION('center_axis',(0.978147600733806,0.20791169081776,1.58957929685218E-15));
#133438=DIRECTION('ref_axis',(0.20791169081776,-0.978147600733806,-6.82961998416069E-15));
#133439=DIRECTION('center_axis',(0.978147600733806,0.207911690817757,4.29175525433417E-15));
#133440=DIRECTION('ref_axis',(0.207911690817757,-0.978147600733806,-6.8296199841607E-15));
#133441=DIRECTION('center_axis',(0.978147600733806,0.20791169081776,1.58957929685218E-15));
#133442=DIRECTION('ref_axis',(0.20791169081776,-0.978147600733806,-6.82961998416069E-15));
#133443=DIRECTION('center_axis',(-0.847105178672008,-0.18009299163103,0.499979330205211));
#133444=DIRECTION('ref_axis',(0.488852904976872,0.104894406038809,0.866036951219426));
#133445=DIRECTION('center_axis',(0.489078846174021,0.103956917928296,-0.866022425483277));
#133446=DIRECTION('ref_axis',(0.870740269393765,-5.71691885207346E-16,0.491743208652721));
#133447=DIRECTION('center_axis',(0.489078854950998,0.103956919793908,-0.866022420302606));
#133448=DIRECTION('ref_axis',(-0.207911690815927,0.978147600734195,1.10148110841986E-12));
#133449=DIRECTION('center_axis',(-0.475533027092007,-0.154510046711426,
-0.866022508720152));
#133450=DIRECTION('ref_axis',(0.30901699437304,-0.951056516295773,1.14519068158217E-12));
#133451=DIRECTION('center_axis',(-0.82364155778377,-0.267585776505831,-0.500012436348634));
#133452=DIRECTION('ref_axis',(0.475234043093109,0.15545353448369,-0.866017784402783));
#133453=DIRECTION('center_axis',(0.475533035318149,0.154510049384265,0.866022503726307));
#133454=DIRECTION('ref_axis',(-0.876548788012431,1.65548636897334E-15,0.481313018974075));
#133455=DIRECTION('center_axis',(0.951056516295146,0.309016994374972,2.15785413849121E-15));
#133456=DIRECTION('ref_axis',(0.309016994374972,-0.951056516295146,-6.82961998416073E-15));
#133457=DIRECTION('center_axis',(-0.951056516295153,-0.309016994374948,
-2.29177897539323E-15));
#133458=DIRECTION('ref_axis',(-0.309016994374948,0.951056516295153,6.82961998416066E-15));
#133459=DIRECTION('center_axis',(-0.951056516295148,-0.309016994374964,
-2.15785413849116E-15));
#133460=DIRECTION('ref_axis',(-0.309016994374964,0.951056516295148,6.82961998416075E-15));
#133461=DIRECTION('center_axis',(-0.951056516295153,-0.309016994374948,
-2.29177897539323E-15));
#133462=DIRECTION('ref_axis',(-0.309016994374948,0.951056516295153,6.82961998416066E-15));
#133463=DIRECTION('center_axis',(0.951056516295165,0.309016994374914,2.15785413849081E-15));
#133464=DIRECTION('ref_axis',(0.309016994374914,-0.951056516295164,-6.82961998416067E-15));
#133465=DIRECTION('center_axis',(-0.503987876168977,-0.163755587629907,
0.848045003637583));
#133466=DIRECTION('ref_axis',(-0.859649462041492,-3.17523175098311E-16,
-0.510884333691858));
#133467=DIRECTION('center_axis',(0.475533164204456,0.154510091262,-0.866022425483259));
#133468=DIRECTION('ref_axis',(0.87654871462881,1.46236813511121E-15,0.481313152617484));
#133469=DIRECTION('center_axis',(0.503987842607937,0.163755599464321,-0.848045021297501));
#133470=DIRECTION('ref_axis',(0.805199544420696,0.266156471007566,0.529919264233244));
#133471=DIRECTION('center_axis',(-0.503987822791217,-0.163755570286421,
0.84804503870864));
#133472=DIRECTION('ref_axis',(-0.859649495083695,-1.02670203161972E-15,
-0.510884278092749));
#133473=DIRECTION('center_axis',(0.475533174128557,0.154510105544451,-0.86602241748575));
#133474=DIRECTION('ref_axis',(0.822222161144199,0.271938812462168,0.500000000000029));
#133475=DIRECTION('center_axis',(0.823661100222806,0.26758748354006,-0.499979330205214));
#133476=DIRECTION('ref_axis',(0.475806237446429,0.153585232133988,0.866036951219416));
#133477=DIRECTION('center_axis',(-0.309247612517368,0.950981553003163,6.64066869178921E-15));
#133478=DIRECTION('ref_axis',(0.950981553003163,0.309247612517368,3.41480999208042E-15));
#133479=DIRECTION('center_axis',(-0.951056516295153,-0.309016994374948,
-2.29177897539323E-15));
#133480=DIRECTION('ref_axis',(-0.309016994374948,0.951056516295153,6.82961998416066E-15));
#133481=DIRECTION('center_axis',(0.951056516295165,0.309016994374914,2.15785413849081E-15));
#133482=DIRECTION('ref_axis',(0.309016994374914,-0.951056516295164,-6.82961998416067E-15));
#133483=DIRECTION('center_axis',(-6.89206998773325E-18,-6.93944786036197E-15,
1.));
#133484=DIRECTION('ref_axis',(0.,-1.,-6.93917548301887E-15));
#133485=DIRECTION('center_axis',(-0.308786358061007,0.95113142366101,6.64171523299944E-15));
#133486=DIRECTION('ref_axis',(0.95113142366101,0.308786358061007,3.41480999208033E-15));
#133487=DIRECTION('center_axis',(0.503988317040591,0.163755730877766,0.848044713969305));
#133488=DIRECTION('ref_axis',(-0.859649189130459,9.85221772351679E-16,0.510884792910637));
#133489=DIRECTION('center_axis',(0.503987822791257,0.163755570286483,-0.848045038708604));
#133490=DIRECTION('ref_axis',(0.859649495083668,-9.8120496246209E-16,0.510884278092794));
#133491=DIRECTION('center_axis',(0.503988355850447,0.163755716975672,0.848044693589287));
#133492=DIRECTION('ref_axis',(-0.805129291879168,-0.266368911010095,0.52991926423319));
#133493=DIRECTION('center_axis',(0.503988379172007,0.163755751065438,0.848044673146744));
#133494=DIRECTION('ref_axis',(-0.859649150669465,-1.91533628641601E-15,
0.510884857627692));
#133495=DIRECTION('center_axis',(-0.503987842737568,-0.163755599577719,
0.848045021198565));
#133496=DIRECTION('ref_axis',(0.807862963765903,0.25795930913596,0.529919264233213));
#133497=DIRECTION('center_axis',(0.503987876169007,0.163755587629917,-0.848045003637563));
#133498=DIRECTION('ref_axis',(0.859649462041474,-1.19924147547379E-15,0.510884333691888));
#133499=DIRECTION('center_axis',(-0.309262527968962,0.950976702550723,2.35377991522115E-14));
#133500=DIRECTION('ref_axis',(0.950976702550723,0.309262527968962,3.4148099920802E-15));
#133501=DIRECTION('center_axis',(0.951056516295148,0.309016994374964,5.41206908565348E-14));
#133502=DIRECTION('ref_axis',(0.309016994374964,-0.951056516295148,-6.82961998416119E-15));
#133503=DIRECTION('center_axis',(-6.89206998773325E-18,-6.93944786036197E-15,
1.));
#133504=DIRECTION('ref_axis',(0.,-1.,-6.93660006688881E-15));
#133505=DIRECTION('center_axis',(-0.308771440182806,0.951136266645025,6.64174905137606E-15));
#133506=DIRECTION('ref_axis',(0.951136266645025,0.308771440182806,3.41480999208035E-15));
#133507=DIRECTION('center_axis',(0.951056516295153,0.309016994374948,2.29177897539323E-15));
#133508=DIRECTION('ref_axis',(0.309016994374948,-0.951056516295153,-6.82961998416059E-15));
#133509=DIRECTION('center_axis',(0.823622990673535,0.267642920194618,0.500012436349017));
#133510=DIRECTION('ref_axis',(0.475845712147552,0.153571010705906,-0.866017784402581));
#133511=DIRECTION('center_axis',(-0.503988379172001,-0.163755751065509,
-0.848044673146734));
#133512=DIRECTION('ref_axis',(0.859649150669465,1.85736175073367E-15,-0.510884857627692));
#133513=DIRECTION('center_axis',(-0.475533025685126,-0.154510035619843,
-0.866022511471558));
#133514=DIRECTION('ref_axis',(-0.825011387616483,-0.263355672623859,0.49999999999996));
#133515=DIRECTION('center_axis',(0.475533035318008,0.154510049384242,0.866022503726388));
#133516=DIRECTION('ref_axis',(-0.87654878801251,1.92597280652308E-16,0.481313018973931));
#133517=DIRECTION('center_axis',(-0.50398835568966,-0.16375571684218,-0.848044693710619));
#133518=DIRECTION('ref_axis',(-0.807930997354701,-0.257746148192231,0.529919264233247));
#133519=DIRECTION('center_axis',(-0.50398831704056,-0.163755730877761,-0.848044713969325));
#133520=DIRECTION('ref_axis',(0.859649189130478,3.22133773568149E-16,-0.510884792910605));
#133521=DIRECTION('center_axis',(0.951056516295148,0.309016994374964,5.41206908565348E-14));
#133522=DIRECTION('ref_axis',(0.309016994374964,-0.951056516295148,-6.82961998416119E-15));
#133523=DIRECTION('center_axis',(-0.951056516295148,-0.309016994374964,
-2.15785413849116E-15));
#133524=DIRECTION('ref_axis',(-0.309016994374964,0.951056516295148,6.82961998416075E-15));
#133525=DIRECTION('center_axis',(0.951056516295153,0.309016994374948,2.29177897539323E-15));
#133526=DIRECTION('ref_axis',(0.309016994374948,-0.951056516295153,-6.82961998416059E-15));
#133527=DIRECTION('center_axis',(0.951056516295148,0.309016994374964,-1.47258949833367E-14));
#133528=DIRECTION('ref_axis',(0.309016994374964,-0.951056516295148,-6.82961998416061E-15));
#133529=DIRECTION('center_axis',(0.951056516295153,0.309016994374948,2.29177897539323E-15));
#133530=DIRECTION('ref_axis',(0.309016994374948,-0.951056516295153,-6.82961998416059E-15));
#133531=DIRECTION('center_axis',(-0.823639804208724,-0.267653025932271,
0.499979330205074));
#133532=DIRECTION('ref_axis',(0.475210466544364,0.15541882643076,0.866036951219504));
#133533=DIRECTION('center_axis',(0.475533164204417,0.154510091261987,-0.866022425483283));
#133534=DIRECTION('ref_axis',(0.876548714628833,-9.26574607259983E-16,0.481313152617443));
#133535=DIRECTION('center_axis',(0.475533172743519,0.154510094036525,-0.866022420299444));
#133536=DIRECTION('ref_axis',(-0.309016994369036,0.951056516297074,3.61478125659533E-12));
#133537=DIRECTION('center_axis',(-0.456777309669968,-0.203370361063118,
-0.866022508721178));
#133538=DIRECTION('ref_axis',(0.406736643078441,-0.913545457641425,-1.66970549760595E-12));
#133539=DIRECTION('center_axis',(-0.791159233141002,-0.352213899941929,
-0.500012436348776));
#133540=DIRECTION('ref_axis',(0.456381342238393,0.20427742791317,-0.866017784402758));
#133541=DIRECTION('center_axis',(0.456777317573273,0.203370364581906,0.866022503726311));
#133542=DIRECTION('ref_axis',(-0.884507036382099,-1.20094363058356E-15,
0.466526850878443));
#133543=DIRECTION('center_axis',(0.913545457642594,0.406736643075817,-5.81845465367576E-14));
#133544=DIRECTION('ref_axis',(0.406736643075817,-0.913545457642593,-6.82961998416125E-15));
#133545=DIRECTION('center_axis',(-0.913545457642601,-0.406736643075801,
-2.96886944389428E-15));
#133546=DIRECTION('ref_axis',(-0.406736643075801,0.9135454576426,6.82961998416066E-15));
#133547=DIRECTION('center_axis',(-0.913545457642598,-0.406736643075807,
-2.84022679824576E-15));
#133548=DIRECTION('ref_axis',(-0.406736643075807,0.913545457642598,6.8296199841606E-15));
#133549=DIRECTION('center_axis',(-0.913545457642601,-0.406736643075801,
-2.96886944389428E-15));
#133550=DIRECTION('ref_axis',(-0.406736643075801,0.9135454576426,6.82961998416066E-15));
#133551=DIRECTION('center_axis',(0.913545457642594,0.406736643075817,2.84022679824583E-15));
#133552=DIRECTION('ref_axis',(0.406736643075817,-0.913545457642593,-6.82961998416057E-15));
#133553=DIRECTION('center_axis',(-0.48410985792377,-0.215539595588312,0.848045003637575));
#133554=DIRECTION('ref_axis',(-0.868458021515995,2.11054687512659E-16,-0.495762710240014));
#133555=DIRECTION('center_axis',(0.456777441376059,0.203370419702488,-0.866022425483298));
#133556=DIRECTION('ref_axis',(0.884506966812066,-1.6326678946194E-15,0.466526982779045));
#133557=DIRECTION('center_axis',(0.484109823307075,0.215539603855264,-0.848045021297519));
#133558=DIRECTION('ref_axis',(0.772967650150695,0.348864709042188,0.529919264233168));
#133559=DIRECTION('center_axis',(-0.484109806651296,-0.215539572760336,
0.848045038708639));
#133560=DIRECTION('ref_axis',(-0.868458052949952,3.7813810093915E-16,-0.495762655175215));
#133561=DIRECTION('center_axis',(0.456777449752818,0.20337043494432,-0.866022417485754));
#133562=DIRECTION('ref_axis',(0.789292595944616,0.356394722164874,0.500000000000031));
#133563=DIRECTION('center_axis',(0.791178490090723,0.352217640366536,-0.499979330205153));
#133564=DIRECTION('ref_axis',(0.457145692792613,0.202479170987194,0.866036951219462));
#133565=DIRECTION('center_axis',(-0.406958162070229,0.913446798847323,6.37856490440285E-15));
#133566=DIRECTION('ref_axis',(0.913446798847323,0.406958162070229,3.41480999208031E-15));
#133567=DIRECTION('center_axis',(-0.913545457642601,-0.406736643075801,
-2.96886944389428E-15));
#133568=DIRECTION('ref_axis',(-0.406736643075801,0.9135454576426,6.82961998416066E-15));
#133569=DIRECTION('center_axis',(0.913545457642598,0.406736643075807,2.84022679824576E-15));
#133570=DIRECTION('ref_axis',(0.406736643075807,-0.913545457642598,-6.8296199841606E-15));
#133571=DIRECTION('center_axis',(-1.21742612413517E-17,-6.92568728168955E-15,
1.));
#133572=DIRECTION('ref_axis',(0.,-1.,-6.92507146780948E-15));
#133573=DIRECTION('center_axis',(-0.406515100163544,0.913644062717546,6.37994239064628E-15));
#133574=DIRECTION('ref_axis',(0.913644062717546,0.406515100163544,3.41480999208035E-15));
#133575=DIRECTION('center_axis',(0.48411028140672,0.215539784135058,0.848044713969328));
#133576=DIRECTION('ref_axis',(-0.868457761888286,-1.79355219875376E-15,
0.495763165045558));
#133577=DIRECTION('center_axis',(0.484109806651295,0.215539572760335,-0.84804503870864));
#133578=DIRECTION('ref_axis',(0.868458052949953,8.16837448075292E-17,0.495762655175213));
#133579=DIRECTION('center_axis',(0.484110321456976,0.215539774366318,0.848044693589282));
#133580=DIRECTION('ref_axis',(-0.772875576444115,-0.349068641861079,0.529919264233184));
#133581=DIRECTION('center_axis',(0.484110341087615,0.215539810706669,0.848044673146743));
#133582=DIRECTION('ref_axis',(-0.868457725299269,-6.1342256846168E-16,0.495763229140705));
#133583=DIRECTION('center_axis',(-0.484109823426906,-0.215539603975436,
0.84804502119857));
#133584=DIRECTION('ref_axis',(0.776473315750794,0.340990855187512,0.5299192642332));
#133585=DIRECTION('center_axis',(0.484109857923801,0.215539595588326,-0.848045003637554));
#133586=DIRECTION('ref_axis',(0.868458021515976,-2.74972831225249E-15,0.495762710240047));
#133587=DIRECTION('center_axis',(-0.406972488803041,0.913440415876952,6.37852033235898E-15));
#133588=DIRECTION('ref_axis',(0.913440415876952,0.406972488803041,3.41480999208023E-15));
#133589=DIRECTION('center_axis',(0.913545457642598,0.406736643075807,2.84022679824576E-15));
#133590=DIRECTION('ref_axis',(0.406736643075807,-0.913545457642598,-6.8296199841606E-15));
#133591=DIRECTION('center_axis',(-1.21742612413517E-17,-6.92568728168955E-15,
1.));
#133592=DIRECTION('ref_axis',(0.,-1.,-6.92909292395928E-15));
#133593=DIRECTION('center_axis',(-0.406500770236728,0.913650438514067,-1.85795542610555E-14));
#133594=DIRECTION('ref_axis',(0.913650438514067,0.406500770236727,3.41480999208053E-15));
#133595=DIRECTION('center_axis',(0.913545457642601,0.406736643075801,2.96886944389428E-15));
#133596=DIRECTION('ref_axis',(0.406736643075801,-0.913545457642601,-6.82961998416062E-15));
#133597=DIRECTION('center_axis',(0.791134794600465,0.352268789801546,0.500012436349572));
#133598=DIRECTION('ref_axis',(0.457186437809986,0.202469153654735,-0.866017784402232));
#133599=DIRECTION('center_axis',(-0.484110341087606,-0.2155398107067,-0.848044673146741));
#133600=DIRECTION('ref_axis',(0.868457725299272,1.42879581731315E-15,-0.495763229140699));
#133601=DIRECTION('center_axis',(-0.456777309431663,-0.20337034988632,-0.866022511471548));
#133602=DIRECTION('ref_axis',(-0.792963725159232,-0.34815015522271,0.499999999999996));
#133603=DIRECTION('center_axis',(0.456777317573163,0.203370364581857,0.866022503726381));
#133604=DIRECTION('ref_axis',(-0.88450703638216,-2.11081026387279E-15,0.466526850878326));
#133605=DIRECTION('center_axis',(-0.484110321309854,-0.215539774219457,
-0.848044693710594));
#133606=DIRECTION('ref_axis',(-0.776563258035295,-0.34078597339695,0.529919264233242));
#133607=DIRECTION('center_axis',(-0.484110281406723,-0.215539784135059,
-0.848044713969326));
#133608=DIRECTION('ref_axis',(0.868457761888284,1.78019109930865E-15,-0.495763165045561));
#133609=DIRECTION('center_axis',(0.913545457642598,0.406736643075807,2.84022679824576E-15));
#133610=DIRECTION('ref_axis',(0.406736643075807,-0.913545457642598,-6.8296199841606E-15));
#133611=DIRECTION('center_axis',(-0.913545457642598,-0.406736643075807,
-2.84022679824576E-15));
#133612=DIRECTION('ref_axis',(-0.406736643075807,0.913545457642598,6.8296199841606E-15));
#133613=DIRECTION('center_axis',(0.913545457642601,0.406736643075801,2.96886944389428E-15));
#133614=DIRECTION('ref_axis',(0.406736643075801,-0.913545457642601,-6.82961998416062E-15));
#133615=DIRECTION('center_axis',(0.913545457642598,0.406736643075807,-1.93826268484815E-14));
#133616=DIRECTION('ref_axis',(0.406736643075807,-0.913545457642598,-6.8296199841606E-15));
#133617=DIRECTION('center_axis',(0.913545457642601,0.406736643075801,2.96886944389428E-15));
#133618=DIRECTION('ref_axis',(0.406736643075801,-0.913545457642601,-6.82961998416062E-15));
#133619=DIRECTION('center_axis',(-0.791150459692754,-0.352280597671016,
0.499979330205255));
#133620=DIRECTION('ref_axis',(0.456361522795892,0.204240445637063,0.866036951219397));
#133621=DIRECTION('center_axis',(0.456777441376069,0.203370419702474,-0.866022425483296));
#133622=DIRECTION('ref_axis',(0.884506966812061,-1.94827188835773E-15,0.466526982779054));
#133623=DIRECTION('center_axis',(0.456777449574972,0.20337042335284,-0.866022420301617));
#133624=DIRECTION('ref_axis',(-0.406736643074073,0.91354545764337,1.08399728130801E-12));
#133625=DIRECTION('center_axis',(-0.43301704445909,-0.250002507182135,-0.866022508720507));
#133626=DIRECTION('ref_axis',(0.500000000001343,-0.866025403783663,-9.13529971196899E-13));
#133627=DIRECTION('center_axis',(-0.750008802378837,-0.432983094185202,
-0.500012436349409));
#133628=DIRECTION('ref_axis',(0.432528431868679,0.250863215167168,-0.866017784402383));
#133629=DIRECTION('center_axis',(0.433017051950287,0.250002511507189,0.866022503726306));
#133630=DIRECTION('ref_axis',(-0.89442479486378,1.23985474967347E-15,0.447218387740135));
#133631=DIRECTION('center_axis',(0.86602540378444,0.499999999999998,6.44677165429795E-14));
#133632=DIRECTION('ref_axis',(0.499999999999998,-0.86602540378444,-6.82961998416156E-15));
#133633=DIRECTION('center_axis',(-0.866025403784438,-0.500000000000001,
-3.61343235749215E-15));
#133634=DIRECTION('ref_axis',(-0.500000000000001,0.866025403784438,6.82961998416066E-15));
#133635=DIRECTION('center_axis',(-0.866025403784433,-0.50000000000001,-3.4914813388432E-15));
#133636=DIRECTION('ref_axis',(-0.50000000000001,0.866025403784433,6.82961998416047E-15));
#133637=DIRECTION('center_axis',(-0.866025403784438,-0.500000000000001,
-3.61343235749215E-15));
#133638=DIRECTION('ref_axis',(-0.500000000000001,0.866025403784438,6.82961998416066E-15));
#133639=DIRECTION('center_axis',(0.86602540378444,0.499999999999998,3.49148133884312E-15));
#133640=DIRECTION('ref_axis',(0.499999999999998,-0.86602540378444,-6.82961998416073E-15));
#133641=DIRECTION('center_axis',(-0.458927830768609,-0.264962106632872,
0.848045003637595));
#133642=DIRECTION('ref_axis',(-0.879478602053341,-1.06564665462097E-15,
-0.475938429348062));
#133643=DIRECTION('center_axis',(0.433017169313211,0.25000257926669,-0.866022425483299));
#133644=DIRECTION('ref_axis',(0.89442473021642,1.22965716892193E-15,0.447218517033098));
#133645=DIRECTION('center_axis',(0.458927795479855,0.26496211123202,-0.848045021297496));
#133646=DIRECTION('ref_axis',(0.73226696056946,0.427750712276335,0.529919264233198));
#133647=DIRECTION('center_axis',(-0.45892778216322,-0.264962078570537,0.848045038708634));
#133648=DIRECTION('ref_axis',(-0.879478631391241,1.07865946136944E-15,-0.475938375135048));
#133649=DIRECTION('center_axis',(0.433017176053256,0.250002595296572,-0.866022417485738));
#133650=DIRECTION('ref_axis',(0.747715375895629,0.436945896707163,0.500000000000031));
#133651=DIRECTION('center_axis',(0.750027562856292,0.432988827019189,-0.499979330205157));
#133652=DIRECTION('ref_axis',(0.433476564270849,0.249154705655846,0.866036951219455));
#133653=DIRECTION('center_axis',(-0.500209992837911,0.865904130412309,6.04657622512354E-15));
#133654=DIRECTION('ref_axis',(0.865904130412309,0.500209992837911,3.41480999208024E-15));
#133655=DIRECTION('center_axis',(-0.866025403784438,-0.500000000000001,
-3.61343235749215E-15));
#133656=DIRECTION('ref_axis',(-0.500000000000001,0.866025403784438,6.82961998416066E-15));
#133657=DIRECTION('center_axis',(0.866025403784433,0.50000000000001,3.4914813388432E-15));
#133658=DIRECTION('ref_axis',(0.50000000000001,-0.866025403784433,-6.82961998416068E-15));
#133659=DIRECTION('center_axis',(-1.88658882409001E-17,-6.91255422424131E-15,
1.));
#133660=DIRECTION('ref_axis',(0.,-1.,-6.91096745260009E-15));
#133661=DIRECTION('center_axis',(-0.499789977759974,0.86614662623062,6.04826956437229E-15));
#133662=DIRECTION('ref_axis',(0.86614662623062,0.499789977759974,3.4148099920803E-15));
#133663=DIRECTION('center_axis',(0.458928232223209,0.264962338412798,0.848044713969318));
#133664=DIRECTION('ref_axis',(-0.879478359737742,1.39963335782071E-15,0.475938877118703));
#133665=DIRECTION('center_axis',(0.458927782163206,0.264962078570538,-0.848045038708641));
#133666=DIRECTION('ref_axis',(0.879478631391249,-4.79831185544794E-17,0.475938375135034));
#133667=DIRECTION('center_axis',(0.458928273074798,0.26496233288458,0.848044693589285));
#133668=DIRECTION('ref_axis',(-0.7321540744614,-0.42794390361835,0.529919264233203));
#133669=DIRECTION('center_axis',(0.458928288799671,0.264962371077201,0.848044673146735));
#133670=DIRECTION('ref_axis',(-0.879478325588501,8.76012990705856E-16,0.475938940222426));
#133671=DIRECTION('center_axis',(-0.458927795588222,-0.264962111360946,
0.848045021198571));
#133672=DIRECTION('ref_axis',(0.736576463603418,0.420286434066109,0.529919264233219));
#133673=DIRECTION('center_axis',(0.458927830768629,0.264962106632892,-0.848045003637579));
#133674=DIRECTION('ref_axis',(0.879478602053329,-1.60404569334003E-16,0.475938429348085));
#133675=DIRECTION('center_axis',(-0.500223573885338,0.86589628485713,-1.76084488451793E-14));
#133676=DIRECTION('ref_axis',(0.86589628485713,0.500223573885338,3.41480999208019E-15));
#133677=DIRECTION('center_axis',(0.866025403784433,0.50000000000001,3.4914813388432E-15));
#133678=DIRECTION('ref_axis',(0.50000000000001,-0.866025403784433,-6.82961998416068E-15));
#133679=DIRECTION('center_axis',(-1.88658882409001E-17,-6.91255422424131E-15,
1.));
#133680=DIRECTION('ref_axis',(0.,-1.,-6.91407863810021E-15));
#133681=DIRECTION('center_axis',(-0.499776392786186,0.866154464985102,2.97103476758308E-14));
#133682=DIRECTION('ref_axis',(0.866154464985102,0.499776392786186,3.41480999208003E-15));
#133683=DIRECTION('center_axis',(0.866025403784438,0.500000000000001,3.61343235749215E-15));
#133684=DIRECTION('ref_axis',(0.500000000000001,-0.866025403784438,-6.82961998416072E-15));
#133685=DIRECTION('center_axis',(0.749978760163145,0.433035128829332,0.500012436349253));
#133686=DIRECTION('ref_axis',(-0.433518133161068,-0.249149002244091,0.866017784402443));
#133687=DIRECTION('center_axis',(-0.458928288799668,-0.264962371077187,
-0.848044673146741));
#133688=DIRECTION('ref_axis',(0.879478325588504,-1.71293817094444E-16,-0.475938940222421));
#133689=DIRECTION('center_axis',(-0.433017045390677,-0.250002496038782,
-0.86602251147156));
#133690=DIRECTION('ref_axis',(-0.752228186194176,-0.429130231858645,0.499999999999966));
#133691=DIRECTION('center_axis',(0.433017051950197,0.250002511507145,0.866022503726364));
#133692=DIRECTION('ref_axis',(-0.894424794863829,1.34326219726227E-15,0.447218387740037));
#133693=DIRECTION('center_axis',(-0.458928272943121,-0.264962332724383,
-0.848044693710595));
#133694=DIRECTION('ref_axis',(-0.73668732915487,-0.420092076165676,0.529919264233218));
#133695=DIRECTION('center_axis',(-0.458928232223181,-0.264962338412827,
-0.848044713969324));
#133696=DIRECTION('ref_axis',(0.879478359737755,-2.53168492317654E-16,-0.475938877118678));
#133697=DIRECTION('center_axis',(0.866025403784433,0.50000000000001,1.71507213071646E-14));
#133698=DIRECTION('ref_axis',(0.50000000000001,-0.866025403784433,-6.82961998416068E-15));
#133699=DIRECTION('center_axis',(-0.866025403784433,-0.50000000000001,-3.4914813388432E-15));
#133700=DIRECTION('ref_axis',(-0.50000000000001,0.866025403784433,6.82961998416068E-15));
#133701=DIRECTION('center_axis',(0.866025403784438,0.500000000000001,3.61343235749215E-15));
#133702=DIRECTION('ref_axis',(0.500000000000001,-0.866025403784438,-6.82961998416072E-15));
#133703=DIRECTION('center_axis',(0.866025403784433,0.50000000000001,3.4914813388432E-15));
#133704=DIRECTION('ref_axis',(0.50000000000001,-0.866025403784433,-6.82961998416068E-15));
#133705=DIRECTION('center_axis',(0.866025403784438,0.500000000000001,3.61343235749215E-15));
#133706=DIRECTION('ref_axis',(0.500000000000001,-0.866025403784438,-6.82961998416072E-15));
#133707=DIRECTION('center_axis',(-0.749993105181594,-0.433048509462309,
0.499979330205302));
#133708=DIRECTION('ref_axis',(-0.4325125867043,-0.250824363778751,-0.866036951219369));
#133709=DIRECTION('center_axis',(0.433017169313192,0.250002579266714,-0.866022425483302));
#133710=DIRECTION('ref_axis',(0.894424730216429,2.21005739164742E-15,0.447218517033081));
#133711=DIRECTION('center_axis',(0.433017177084447,0.250002583753453,-0.866022420302393));
#133712=DIRECTION('ref_axis',(-0.499999999997911,0.866025403785645,1.4118190397783E-12));
#133713=DIRECTION('center_axis',(-0.404512553894144,-0.293895573516168,
-0.866022508719975));
#133714=DIRECTION('ref_axis',(0.587785252291208,-0.809016994375867,9.0915901439341E-13));
#133715=DIRECTION('center_axis',(-0.700641118228567,-0.509008435041749,
-0.500012436349111));
#133716=DIRECTION('ref_axis',(0.403936649451869,0.294700492582192,-0.866017784402498));
#133717=DIRECTION('center_axis',(0.404512560891457,0.293895578600013,0.866022503726317));
#133718=DIRECTION('ref_axis',(-0.906035256115487,1.17177266627819E-15,0.423202214875754));
#133719=DIRECTION('center_axis',(0.809016994374931,0.587785252292496,4.1044824792529E-15));
#133720=DIRECTION('ref_axis',(0.587785252292496,-0.809016994374931,-6.82961998416073E-15));
#133721=DIRECTION('center_axis',(-0.809016994374947,-0.587785252292474,
-4.21840575002201E-15));
#133722=DIRECTION('ref_axis',(-0.587785252292474,0.809016994374947,6.82961998416066E-15));
#133723=DIRECTION('center_axis',(-0.809016994374931,-0.587785252292496,
2.80103167643605E-14));
#133724=DIRECTION('ref_axis',(-0.587785252292496,0.809016994374931,6.82961998416073E-15));
#133725=DIRECTION('center_axis',(-0.809016994374947,-0.587785252292474,
-4.21840575002201E-15));
#133726=DIRECTION('ref_axis',(-0.587785252292474,0.809016994374947,6.82961998416066E-15));
#133727=DIRECTION('center_axis',(0.80901699437495,0.58778525229247,4.10448247925272E-15));
#133728=DIRECTION('ref_axis',(0.58778525229247,-0.80901699437495,-6.82961998416043E-15));
#133729=DIRECTION('center_axis',(-0.428717694262756,-0.311481637390317,
0.848045003637586));
#133730=DIRECTION('ref_axis',(-0.892442058026272,-3.95378541852584E-16,
-0.45116202529228));
#133731=DIRECTION('center_axis',(0.404512670528671,0.293895658256124,-0.866022425483291));
#133732=DIRECTION('ref_axis',(0.906035197473499,1.39606431300021E-15,0.423202340422591));
#133733=DIRECTION('center_axis',(0.428717658681342,0.311481638282739,-0.848045021297507));
#133734=DIRECTION('ref_axis',(0.683543400919793,0.501950189215568,0.529919264233203));
#133735=DIRECTION('center_axis',(-0.428717648856913,-0.31148160440104,0.848045038708649));
#133736=DIRECTION('ref_axis',(-0.892442084777739,-1.07749458524948E-15,
-0.451161972375291));
#133737=DIRECTION('center_axis',(0.404512675554594,0.293895674904847,-0.866022417485765));
#133738=DIRECTION('ref_axis',(0.697946029716722,0.51270980057208,0.500000000000003));
#133739=DIRECTION('center_axis',(0.700659176689849,0.509016097474139,-0.49997933020526));
#133740=DIRECTION('ref_axis',(0.405058175792274,0.293100449242975,0.866036951219404));
#133741=DIRECTION('center_axis',(-0.587981418248406,0.808874435122407,-7.06716172179891E-14));
#133742=DIRECTION('ref_axis',(0.808874435122407,0.587981418248406,3.41480999207993E-15));
#133743=DIRECTION('center_axis',(-0.809016994374947,-0.587785252292474,
-4.21840575002201E-15));
#133744=DIRECTION('ref_axis',(-0.587785252292474,0.809016994374947,6.82961998416066E-15));
#133745=DIRECTION('center_axis',(0.809016994374969,0.587785252292444,4.10448247925254E-15));
#133746=DIRECTION('ref_axis',(0.587785252292444,-0.809016994374969,-6.8296199841606E-15));
#133747=DIRECTION('center_axis',(-2.68936361206584E-17,-6.90019257654293E-15,
1.));
#133748=DIRECTION('ref_axis',(0.,-1.,-6.8968634373907E-15));
#133749=DIRECTION('center_axis',(-0.587589051772239,0.809159506053906,5.65033063106948E-15));
#133750=DIRECTION('ref_axis',(0.809159506053906,0.587589051772239,3.41480999208021E-15));
#133751=DIRECTION('center_axis',(0.428718069290544,0.311481909863913,0.848044713969327));
#133752=DIRECTION('ref_axis',(-0.892441837073393,-4.22102850772109E-15,
0.451162462358148));
#133753=DIRECTION('center_axis',(0.428717648856975,0.311481604401142,-0.848045038708581));
#133754=DIRECTION('ref_axis',(0.892442084777698,3.18562187189916E-15,0.451161972375372));
#133755=DIRECTION('center_axis',(0.428718110493366,0.311481908639993,0.848044693589309));
#133756=DIRECTION('ref_axis',(-0.683410939232418,-0.502130522406281,0.529919264233204));
#133757=DIRECTION('center_axis',(0.428718122142701,0.311481948263281,0.848044673146731));
#133758=DIRECTION('ref_axis',(-0.892441805934775,3.97758164497583E-16,0.451162523953261));
#133759=DIRECTION('center_axis',(-0.428717658777612,-0.311481638419594,
0.848045021198573));
#133760=DIRECTION('ref_axis',(0.688609525573209,0.494977266835898,0.529919264233246));
#133761=DIRECTION('center_axis',(0.428717694262811,0.311481637390356,-0.848045003637544));
#133762=DIRECTION('ref_axis',(0.892442058026239,2.8004224903515E-15,0.451162025292345));
#133763=DIRECTION('center_axis',(-0.587994104813606,0.808865212939984,5.64827559323867E-15));
#133764=DIRECTION('ref_axis',(0.808865212939984,0.587994104813606,3.41480999208028E-15));
#133765=DIRECTION('center_axis',(0.809016994374931,0.587785252292496,8.04215107813387E-14));
#133766=DIRECTION('ref_axis',(0.587785252292496,-0.809016994374931,-6.82961998416074E-15));
#133767=DIRECTION('center_axis',(-2.68936361206584E-17,-6.90019257654293E-15,
1.));
#133768=DIRECTION('ref_axis',(0.,-1.,-6.89906435224115E-15));
#133769=DIRECTION('center_axis',(-0.587576360591353,0.80916872188328,3.77537810209823E-14));
#133770=DIRECTION('ref_axis',(0.80916872188328,0.587576360591353,3.41480999207978E-15));
#133771=DIRECTION('center_axis',(0.809016994374947,0.587785252292474,4.21840575002201E-15));
#133772=DIRECTION('ref_axis',(0.587785252292474,-0.809016994374947,-6.82961998416063E-15));
#133773=DIRECTION('center_axis',(0.700605801485416,0.509057044367926,0.500012436349707));
#133774=DIRECTION('ref_axis',(-0.405100113157865,-0.29309912217315,0.866017784402153));
#133775=DIRECTION('center_axis',(-0.428718122142726,-0.311481948263249,
-0.848044673146731));
#133776=DIRECTION('ref_axis',(0.892441805934765,-1.92098507058835E-15,-0.451162523953281));
#133777=DIRECTION('center_axis',(-0.404512555979938,-0.293895562537369,
-0.86602251147151));
#133778=DIRECTION('ref_axis',(-0.703251077800027,-0.505408667884764,0.500000000000049));
#133779=DIRECTION('center_axis',(0.404512560891371,0.293895578599951,0.866022503726378));
#133780=DIRECTION('ref_axis',(-0.906035256115534,2.25474787958917E-15,0.423202214875655));
#133781=DIRECTION('center_axis',(-0.428718110383991,-0.311481908460264,
-0.848044693710616));
#133782=DIRECTION('ref_axis',(-0.688740099734959,-0.494795562239232,0.529919264233185));
#133783=DIRECTION('center_axis',(-0.428718069290536,-0.311481909863907,
-0.848044713969333));
#133784=DIRECTION('ref_axis',(0.892441837073399,-2.5998686034382E-15,-0.451162462358136));
#133785=DIRECTION('center_axis',(0.809016994374931,0.587785252292496,4.1044824792529E-15));
#133786=DIRECTION('ref_axis',(0.587785252292496,-0.809016994374931,-6.82961998416073E-15));
#133787=DIRECTION('center_axis',(-0.80901699437495,-0.58778525229247,-4.10448247925272E-15));
#133788=DIRECTION('ref_axis',(-0.58778525229247,0.80901699437495,6.82961998416043E-15));
#133789=DIRECTION('center_axis',(0.809016994374947,0.587785252292474,4.21840575002201E-15));
#133790=DIRECTION('ref_axis',(0.587785252292474,-0.809016994374947,-6.82961998416063E-15));
#133791=DIRECTION('center_axis',(0.809016994374931,0.587785252292496,4.83067115377211E-14));
#133792=DIRECTION('ref_axis',(0.587785252292496,-0.809016994374931,-6.82961998416074E-15));
#133793=DIRECTION('center_axis',(0.809016994374947,0.587785252292474,4.21840575002201E-15));
#133794=DIRECTION('ref_axis',(0.587785252292474,-0.809016994374947,-6.82961998416063E-15));
#133795=DIRECTION('center_axis',(-0.700618669263898,-0.50907185116288,0.499979330205243));
#133796=DIRECTION('ref_axis',(-0.403924952204111,-0.294660197701536,-0.866036951219403));
#133797=DIRECTION('center_axis',(0.404512670528677,0.293895658256128,-0.866022425483287));
#133798=DIRECTION('ref_axis',(0.906035197473496,1.03251279233693E-15,0.423202340422597));
#133799=DIRECTION('center_axis',(0.404512677787197,0.293895663529747,-0.866022420303217));
#133800=DIRECTION('ref_axis',(-0.587785252301584,0.809016994368328,-6.47338699048409E-12));
#133801=DIRECTION('center_axis',(-0.371576139139117,-0.334568658445484,
-0.866022508719292));
#133802=DIRECTION('ref_axis',(0.669130606356112,-0.743144825479867,2.18984935677441E-12));
#133803=DIRECTION('center_axis',(-0.643597063368043,-0.579456972968032,
-0.500012436348095));
#133804=DIRECTION('ref_axis',(0.370919252614423,0.335308969664565,-0.866017784403095));
#133805=DIRECTION('center_axis',(0.371576145565852,0.334568664232078,0.866022503726311));
#133806=DIRECTION('ref_axis',(-0.918982183096513,9.95361655628204E-19,0.394299058014558));
#133807=DIRECTION('center_axis',(0.743144825477406,0.669130606358845,8.1834950149964E-14));
#133808=DIRECTION('ref_axis',(0.669130606358845,-0.743144825477406,-6.82961998416065E-15));
#133809=DIRECTION('center_axis',(-0.743144825477393,-0.669130606358859,
-4.77716140639646E-15));
#133810=DIRECTION('ref_axis',(-0.669130606358859,0.743144825477393,6.82961998416066E-15));
#133811=DIRECTION('center_axis',(-0.743144825477406,-0.669130606358845,
-4.6725140507014E-15));
#133812=DIRECTION('ref_axis',(-0.669130606358845,0.743144825477406,6.82961998416065E-15));
#133813=DIRECTION('center_axis',(-0.743144825477393,-0.669130606358859,
-4.77716140639646E-15));
#133814=DIRECTION('ref_axis',(-0.669130606358859,0.743144825477393,6.82961998416066E-15));
#133815=DIRECTION('center_axis',(0.743144825477382,0.669130606358872,4.67251405070159E-15));
#133816=DIRECTION('ref_axis',(0.669130606358872,-0.743144825477382,-6.82961998416048E-15));
#133817=DIRECTION('center_axis',(-0.393810436983632,-0.354588510146755,
0.848045003637582));
#133818=DIRECTION('ref_axis',(-0.906978223357768,3.01844662600193E-15,-0.421177518814558));
#133819=DIRECTION('center_axis',(0.371576246276125,0.334568754912027,-0.86602242548329));
#133820=DIRECTION('ref_axis',(0.918982131463642,-2.65789370359083E-15,0.394299178353875));
#133821=DIRECTION('center_axis',(0.393810401511434,0.354588507306632,-0.848045021297488));
#133822=DIRECTION('ref_axis',(0.627330796743794,0.570650194822807,0.529919264233231));
#133823=DIRECTION('center_axis',(-0.393810395274862,-0.35458847259201,0.84804503870863));
#133824=DIRECTION('ref_axis',(-0.906978247051284,-1.28220563798849E-15,
-0.421177467792117));
#133825=DIRECTION('center_axis',(0.371576249535771,0.334568771993211,-0.866022417485763));
#133826=DIRECTION('ref_axis',(0.640529840778939,0.582856348572902,0.499999999999971));
#133827=DIRECTION('center_axis',(0.643614221961138,0.579466481046779,-0.499979330205382));
#133828=DIRECTION('ref_axis',(0.372201885199337,0.33383492294369,0.866036951219312));
#133829=DIRECTION('center_axis',(-0.669310796197597,0.742982542253409,5.18821936272801E-15));
#133830=DIRECTION('ref_axis',(0.742982542253409,0.669310796197597,3.41480999208022E-15));
#133831=DIRECTION('center_axis',(-0.743144825477393,-0.669130606358859,
-4.77716140639646E-15));
#133832=DIRECTION('ref_axis',(-0.669130606358859,0.743144825477393,6.82961998416066E-15));
#133833=DIRECTION('center_axis',(0.743144825477382,0.669130606358872,4.67251405070159E-15));
#133834=DIRECTION('ref_axis',(0.669130606358872,-0.743144825477382,-6.82961998416048E-15));
#133835=DIRECTION('center_axis',(-3.61695511949416E-17,-6.88873777539344E-15,
1.));
#133836=DIRECTION('ref_axis',(0.,-1.,-6.88981142978601E-15));
#133837=DIRECTION('center_axis',(-0.668950377172406,0.743307065001333,5.19048549296483E-15));
#133838=DIRECTION('ref_axis',(0.743307065001333,0.668950377172406,3.41480999208041E-15));
#133839=DIRECTION('center_axis',(0.393810781475684,0.354588820328814,0.848044713969335));
#133840=DIRECTION('ref_axis',(-0.906978027661853,8.31337327814796E-16,0.421177940232647));
#133841=DIRECTION('center_axis',(0.39381039527486,0.354588472592008,-0.848045038708632));
#133842=DIRECTION('ref_axis',(0.906978247051285,2.28558738914555E-15,0.421177467792114));
#133843=DIRECTION('center_axis',(0.393810822584926,0.354588823413865,0.848044693589292));
#133844=DIRECTION('ref_axis',(-0.627180210713234,-0.570815694146828,0.529919264233126));
#133845=DIRECTION('center_axis',(0.393810830024562,0.354588864042297,0.848044673146739));
#133846=DIRECTION('ref_axis',(-0.906978000082633,2.36717991127537E-15,0.421177999622615));
#133847=DIRECTION('center_axis',(-0.393810401582745,-0.354588507464037,
0.848045021198559));
#133848=DIRECTION('ref_axis',(0.633098037497121,0.564245025066081,0.529919264233215));
#133849=DIRECTION('center_axis',(0.393810436983644,0.354588510146766,-0.848045003637571));
#133850=DIRECTION('ref_axis',(0.90697822335776,3.0270894602194E-15,0.421177518814575));
#133851=DIRECTION('center_axis',(-0.6693224492839,0.74297204448391,-3.13815977466195E-14));
#133852=DIRECTION('ref_axis',(0.74297204448391,0.6693224492839,3.41480999208017E-15));
#133853=DIRECTION('center_axis',(0.743144825477406,0.669130606358845,-3.18867480389152E-14));
#133854=DIRECTION('ref_axis',(0.669130606358845,-0.743144825477406,-6.82961998416065E-15));
#133855=DIRECTION('center_axis',(-3.61695511949416E-17,-6.88873777539344E-15,
1.));
#133856=DIRECTION('ref_axis',(0.,-1.,-6.89155720931161E-15));
#133857=DIRECTION('center_axis',(-0.668938718831589,0.743317556935091,5.19055875774668E-15));
#133858=DIRECTION('ref_axis',(0.743317556935091,0.668938718831589,3.41480999208028E-15));
#133859=DIRECTION('center_axis',(0.743144825477393,0.669130606358859,4.77716140639646E-15));
#133860=DIRECTION('ref_axis',(0.669130606358859,-0.743144825477393,-6.82961998416078E-15));
#133861=DIRECTION('center_axis',(0.643556859036851,0.579501624400588,0.500012436349041));
#133862=DIRECTION('ref_axis',(-0.372243731524368,-0.333837986812962,0.866017784402539));
#133863=DIRECTION('center_axis',(-0.393810830024468,-0.35458886404239,-0.848044673146743));
#133864=DIRECTION('ref_axis',(0.906978000082671,3.73207792763548E-15,-0.421177999622533));
#133865=DIRECTION('center_axis',(-0.371576142364556,-0.334568647739141,
-0.866022511471542));
#133866=DIRECTION('ref_axis',(-0.646569003445698,-0.576149740764733,0.499999999999968));
#133867=DIRECTION('center_axis',(0.371576145565767,0.334568664232001,0.866022503726377));
#133868=DIRECTION('ref_axis',(-0.918982183096556,1.80129298120473E-15,0.394299058014457));
#133869=DIRECTION('center_axis',(-0.393810822488479,-0.354588823230846,
-0.848044693710603));
#133870=DIRECTION('ref_axis',(-0.633246889645983,-0.564077964600818,0.529919264233229));
#133871=DIRECTION('center_axis',(-0.393810781475669,-0.354588820328858,
-0.848044713969324));
#133872=DIRECTION('ref_axis',(0.906978027661857,3.69392270454927E-16,-0.421177940232639));
#133873=DIRECTION('center_axis',(0.743144825477406,0.669130606358845,-3.18867480389132E-14));
#133874=DIRECTION('ref_axis',(0.669130606358845,-0.743144825477406,-6.82961998416065E-15));
#133875=DIRECTION('center_axis',(-0.743144825477406,-0.669130606358845,
-4.6725140507014E-15));
#133876=DIRECTION('ref_axis',(-0.669130606358845,0.743144825477406,6.82961998416065E-15));
#133877=DIRECTION('center_axis',(0.743144825477393,0.669130606358859,4.77716140639646E-15));
#133878=DIRECTION('ref_axis',(0.669130606358859,-0.743144825477393,-6.82961998416078E-15));
#133879=DIRECTION('center_axis',(0.743144825477406,0.669130606358845,-3.59306599589443E-14));
#133880=DIRECTION('ref_axis',(0.669130606358845,-0.743144825477406,-6.82961998416065E-15));
#133881=DIRECTION('center_axis',(0.743144825477393,0.669130606358859,4.77716140639646E-15));
#133882=DIRECTION('ref_axis',(0.669130606358859,-0.743144825477393,-6.82961998416078E-15));
#133883=DIRECTION('center_axis',(-0.643568108591872,-0.579517695131965,
0.499979330205175));
#133884=DIRECTION('ref_axis',(-0.370911831410088,-0.335267672826545,-0.866036951219454));
#133885=DIRECTION('center_axis',(0.371576246276117,0.33456875491202,-0.866022425483296));
#133886=DIRECTION('ref_axis',(0.918982131463646,-1.62026352763753E-15,0.394299178353866));
#133887=DIRECTION('center_axis',(0.371576252946869,0.334568760918362,-0.86602242030072));
#133888=DIRECTION('ref_axis',(-0.669130606356659,0.743144825479374,1.67407644653007E-12));
#133889=DIRECTION('center_axis',(-0.334568658443055,-0.371576139136519,
-0.866022508721346));
#133890=DIRECTION('ref_axis',(0.74314482547367,-0.669130606362995,3.24324994554054E-12));
#133891=DIRECTION('center_axis',(-0.579501624401049,-0.643556859036431,
-0.500012436349046));
#133892=DIRECTION('ref_axis',(0.333837986817552,0.372243731520247,-0.866017784402541));
#133893=DIRECTION('center_axis',(0.334568664232049,0.371576145565878,0.866022503726311));
#133894=DIRECTION('ref_axis',(1.29773672876362E-15,-0.918982183096502,0.394299058014582));
#133895=DIRECTION('center_axis',(0.669130606358845,0.743144825477406,5.1893525804244E-15));
#133896=DIRECTION('ref_axis',(0.743144825477406,-0.669130606358845,-3.41480999208033E-15));
#133897=DIRECTION('center_axis',(-0.669130606358857,-0.743144825477395,
-5.28357748271715E-15));
#133898=DIRECTION('ref_axis',(-0.743144825477395,0.669130606358857,3.41480999208033E-15));
#133899=DIRECTION('center_axis',(-0.669130606358845,-0.743144825477406,
-5.1893525804244E-15));
#133900=DIRECTION('ref_axis',(-0.743144825477406,0.669130606358845,3.41480999208033E-15));
#133901=DIRECTION('center_axis',(-0.669130606358857,-0.743144825477395,
-5.28357748271715E-15));
#133902=DIRECTION('ref_axis',(-0.743144825477395,0.669130606358857,3.41480999208033E-15));
#133903=DIRECTION('center_axis',(0.669130606358872,0.743144825477382,5.18935258042423E-15));
#133904=DIRECTION('ref_axis',(0.743144825477382,-0.669130606358872,-3.41480999208052E-15));
#133905=DIRECTION('center_axis',(-0.354588510146771,-0.393810436983662,
0.84804500363756));
#133906=DIRECTION('ref_axis',(-1.78940208541438E-15,-0.90697822335775,-0.421177518814595));
#133907=DIRECTION('center_axis',(0.334568754912014,0.371576246276123,-0.866022425483296));
#133908=DIRECTION('ref_axis',(-1.52738427012904E-15,0.918982131463644,0.394299178353872));
#133909=DIRECTION('center_axis',(0.354588475163086,0.39381043045359,-0.848045021297499));
#133910=DIRECTION('ref_axis',(0.564245025059182,0.63309803750328,0.529919264233202));
#133911=DIRECTION('center_axis',(-0.354588472592013,-0.393810395274878,
0.848045038708622));
#133912=DIRECTION('ref_axis',(-1.03488258956407E-15,-0.906978247051276,
-0.421177467792134));
#133913=DIRECTION('center_axis',(0.334568756368539,0.371576263604268,-0.866022417485772));
#133914=DIRECTION('ref_axis',(0.57609587287146,0.646617000441915,0.499999999999971));
#133915=DIRECTION('center_axis',(0.579517695131787,0.643568108591975,-0.499979330205249));
#133916=DIRECTION('ref_axis',(0.335267672846325,0.37091183139236,0.86603695121939));
#133917=DIRECTION('center_axis',(-0.743307065001336,0.668950377172403,4.67125551701904E-15));
#133918=DIRECTION('ref_axis',(0.668950377172402,0.743307065001336,6.82961998416069E-15));
#133919=DIRECTION('center_axis',(-0.669130606358857,-0.743144825477395,
-5.28357748271715E-15));
#133920=DIRECTION('ref_axis',(-0.743144825477395,0.669130606358857,3.41480999208033E-15));
#133921=DIRECTION('center_axis',(0.669130606358872,0.743144825477382,5.18935258042423E-15));
#133922=DIRECTION('ref_axis',(0.743144825477382,-0.669130606358872,-3.41480999208052E-15));
#133923=DIRECTION('center_axis',(-4.6592004597086E-17,-6.8783153219913E-15,
1.));
#133924=DIRECTION('ref_axis',(0.,-1.,-6.87570741457662E-15));
#133925=DIRECTION('center_axis',(-0.742982542253406,0.669310796197601,4.67377230962033E-15));
#133926=DIRECTION('ref_axis',(0.669310796197601,0.742982542253406,6.82961998416052E-15));
#133927=DIRECTION('center_axis',(0.354588820328813,0.393810781475708,0.848044713969324));
#133928=DIRECTION('ref_axis',(1.92894670706085E-15,-0.906978027661841,0.421177940232672));
#133929=DIRECTION('center_axis',(0.354588472591992,0.393810395274855,-0.848045038708641));
#133930=DIRECTION('ref_axis',(2.31305154500925E-15,0.906978247051289,0.421177467792106));
#133931=DIRECTION('center_axis',(0.354588860892955,0.393810788838664,0.848044693589262));
#133932=DIRECTION('ref_axis',(-0.564077964589757,-0.633246889655851,0.529919264233211));
#133933=DIRECTION('center_axis',(0.354588864042362,0.393810830024493,0.848044673146744));
#133934=DIRECTION('ref_axis',(-1.94575173309401E-15,-0.906978000082661,
0.421177999622554));
#133935=DIRECTION('center_axis',(-0.354588475221977,-0.393810430613613,
0.848045021198565));
#133936=DIRECTION('ref_axis',(0.570650194822096,0.627330796744435,0.529919264233239));
#133937=DIRECTION('center_axis',(0.35458851014676,0.39381043698365,-0.848045003637571));
#133938=DIRECTION('ref_axis',(3.38703812945195E-15,0.906978223357757,0.42117751881458));
#133939=DIRECTION('center_axis',(-0.743317556935091,0.668938718831589,4.67117410726026E-15));
#133940=DIRECTION('ref_axis',(0.668938718831589,0.743317556935091,6.82961998416059E-15));
#133941=DIRECTION('center_axis',(0.669130606358845,0.743144825477406,5.1893525804244E-15));
#133942=DIRECTION('ref_axis',(0.743144825477406,-0.669130606358845,-3.41480999208033E-15));
#133943=DIRECTION('center_axis',(-4.6592004597086E-17,-6.8783153219913E-15,
1.));
#133944=DIRECTION('ref_axis',(0.,-1.,-6.87654292345255E-15));
#133945=DIRECTION('center_axis',(-0.742972044483927,0.669322449283882,6.49863705058621E-16));
#133946=DIRECTION('ref_axis',(0.669322449283881,0.742972044483927,6.82961998416067E-15));
#133947=DIRECTION('center_axis',(0.669130606358857,0.743144825477395,5.28357748271715E-15));
#133948=DIRECTION('ref_axis',(0.743144825477395,-0.669130606358857,-3.41480999208041E-15));
#133949=DIRECTION('center_axis',(0.579456972966333,0.643597063368587,0.500012436349362));
#133950=DIRECTION('ref_axis',(-0.335308969659004,-0.370919252621144,0.86601778440237));
#133951=DIRECTION('center_axis',(-0.354588864042302,-0.393810830024557,
-0.848044673146739));
#133952=DIRECTION('ref_axis',(-1.8722112353852E-15,0.906978000082635,-0.421177999622611));
#133953=DIRECTION('center_axis',(-0.334568662772281,-0.371576128828631,
-0.866022511471553));
#133954=DIRECTION('ref_axis',(-0.582802983775234,-0.640578396531379,0.499999999999971));
#133955=DIRECTION('center_axis',(0.334568664232006,0.37157614556576,0.866022503726378));
#133956=DIRECTION('ref_axis',(1.39319519318679E-15,-0.918982183096559,0.39429905801445));
#133957=DIRECTION('center_axis',(-0.354588860821328,-0.393810788641775,
-0.848044693710641));
#133958=DIRECTION('ref_axis',(-0.570815694135724,-0.627180210723296,0.529919264233179));
#133959=DIRECTION('center_axis',(-0.354588820328737,-0.393810781475754,
-0.848044713969335));
#133960=DIRECTION('ref_axis',(2.97237289164332E-15,0.906978027661824,-0.421177940232709));
#133961=DIRECTION('center_axis',(0.669130606358845,0.743144825477406,9.23326450045792E-15));
#133962=DIRECTION('ref_axis',(0.743144825477406,-0.669130606358845,-3.41480999208032E-15));
#133963=DIRECTION('center_axis',(-0.669130606358875,-0.743144825477379,
-5.18935258042421E-15));
#133964=DIRECTION('ref_axis',(-0.743144825477379,0.669130606358875,3.41480999208015E-15));
#133965=DIRECTION('center_axis',(0.669130606358857,0.743144825477395,5.28357748271715E-15));
#133966=DIRECTION('ref_axis',(0.743144825477395,-0.669130606358857,-3.41480999208041E-15));
#133967=DIRECTION('center_axis',(0.669130606358845,0.743144825477406,5.1893525804244E-15));
#133968=DIRECTION('ref_axis',(0.743144825477406,-0.669130606358845,-3.41480999208033E-15));
#133969=DIRECTION('center_axis',(0.669130606358857,0.743144825477395,5.28357748271715E-15));
#133970=DIRECTION('ref_axis',(0.743144825477395,-0.669130606358857,-3.41480999208041E-15));
#133971=DIRECTION('center_axis',(-0.579466481046696,-0.64361422196136,0.499979330205192));
#133972=DIRECTION('ref_axis',(-0.333834922952809,-0.372201885190879,-0.866036951219431));
#133973=DIRECTION('center_axis',(0.334568754912021,0.371576246276131,-0.86602242548329));
#133974=DIRECTION('ref_axis',(-2.58413282129854E-15,0.91898213146364,0.39429917835388));
#133975=DIRECTION('center_axis',(0.334568760922057,0.371576252950874,-0.866022420297574));
#133976=DIRECTION('ref_axis',(-0.743144825476543,0.669130606359804,6.94982127933865E-13));
#133977=DIRECTION('center_axis',(-0.293895573516141,-0.404512553894111,
-0.86602250872));
#133978=DIRECTION('ref_axis',(0.809016994375186,-0.587785252292144,-2.31660710397836E-13));
#133979=DIRECTION('center_axis',(-0.509057044366969,-0.70060580148708,-0.50001243634835));
#133980=DIRECTION('ref_axis',(0.293099122185064,0.405100113147538,-0.866017784402951));
#133981=DIRECTION('center_axis',(0.293895578600017,0.404512560891464,0.866022503726313));
#133982=DIRECTION('ref_axis',(1.58451773583043E-15,-0.906035256115484,0.42320221487576));
#133983=DIRECTION('center_axis',(0.587785252292434,0.809016994374976,5.64933547733438E-15));
#133984=DIRECTION('ref_axis',(0.809016994374976,-0.587785252292434,-3.41480999208033E-15));
#133985=DIRECTION('center_axis',(-0.587785252292471,-0.809016994374949,
-5.73210557847752E-15));
#133986=DIRECTION('ref_axis',(-0.809016994374949,0.587785252292471,3.41480999208033E-15));
#133987=DIRECTION('center_axis',(-0.587785252292496,-0.809016994374931,
-5.64933547733406E-15));
#133988=DIRECTION('ref_axis',(-0.809016994374931,0.587785252292496,3.41480999208037E-15));
#133989=DIRECTION('center_axis',(-0.587785252292471,-0.809016994374949,
-5.73210557847752E-15));
#133990=DIRECTION('ref_axis',(-0.809016994374949,0.587785252292471,3.41480999208033E-15));
#133991=DIRECTION('center_axis',(0.58778525229247,0.80901699437495,5.6493354773342E-15));
#133992=DIRECTION('ref_axis',(0.80901699437495,-0.58778525229247,-3.41480999208022E-15));
#133993=DIRECTION('center_axis',(-0.311481637390324,-0.428717694262781,
0.848045003637571));
#133994=DIRECTION('ref_axis',(1.27173423926985E-15,-0.892442058026259,-0.451162025292307));
#133995=DIRECTION('center_axis',(0.293895658256083,0.404512670528694,-0.866022425483294));
#133996=DIRECTION('ref_axis',(8.91224751768462E-16,0.90603519747349,0.423202340422609));
#133997=DIRECTION('center_axis',(0.311481603280417,0.42871768411203,-0.848045021297501));
#133998=DIRECTION('ref_axis',(0.49497726682106,0.688609525583905,0.529919264233205));
#133999=DIRECTION('center_axis',(-0.31148160440103,-0.428717648856912,0.848045038708654));
#134000=DIRECTION('ref_axis',(-1.86658406301952E-15,-0.89244208477774,-0.451161972375289));
#134001=DIRECTION('center_axis',(0.293895657889663,0.404512687916895,-0.866022417485743));
#134002=DIRECTION('ref_axis',(0.50535007802797,0.703293181139326,0.500000000000052));
#134003=DIRECTION('center_axis',(0.50907185116279,0.700618669263949,-0.499979330205263));
#134004=DIRECTION('ref_axis',(0.294660197700626,0.403924952204797,0.866036951219393));
#134005=DIRECTION('center_axis',(-0.809159506053914,0.587589051772227,4.10311241834253E-15));
#134006=DIRECTION('ref_axis',(0.587589051772227,0.809159506053914,6.82961998416088E-15));
#134007=DIRECTION('center_axis',(-0.587785252292471,-0.809016994374949,
-5.73210557847752E-15));
#134008=DIRECTION('ref_axis',(-0.809016994374949,0.587785252292471,3.41480999208033E-15));
#134009=DIRECTION('center_axis',(0.58778525229246,0.809016994374957,5.64933547733425E-15));
#134010=DIRECTION('ref_axis',(0.809016994374957,-0.58778525229246,-3.41480999208051E-15));
#134011=DIRECTION('center_axis',(-5.8046805746579E-17,-6.86903940691701E-15,
1.));
#134012=DIRECTION('ref_axis',(0.,-1.,-6.86865540697193E-15));
#134013=DIRECTION('center_axis',(-0.808874435122371,0.587981418248456,4.10585229880201E-15));
#134014=DIRECTION('ref_axis',(0.587981418248456,0.808874435122371,6.82961998416081E-15));
#134015=DIRECTION('center_axis',(0.311481909863959,0.428718069290514,0.848044713969325));
#134016=DIRECTION('ref_axis',(2.35220027834147E-15,-0.892441837073406,0.451162462358122));
#134017=DIRECTION('center_axis',(0.311481604401026,0.428717648856907,-0.848045038708658));
#134018=DIRECTION('ref_axis',(2.02341423291377E-15,0.892442084777743,0.451161972375283));
#134019=DIRECTION('center_axis',(0.311481949432559,0.428718080855898,0.848044693589276));
#134020=DIRECTION('ref_axis',(-0.494795562222334,-0.688740099747117,0.529919264233162));
#134021=DIRECTION('center_axis',(0.311481948263326,0.428718122142669,0.848044673146731));
#134022=DIRECTION('ref_axis',(-1.24965575049336E-15,-0.892441805934789,
0.451162523953235));
#134023=DIRECTION('center_axis',(-0.311481603316802,-0.428717684281317,
0.848045021198556));
#134024=DIRECTION('ref_axis',(0.501950189217994,0.683543400918034,0.529919264233174));
#134025=DIRECTION('center_axis',(0.311481637390342,0.428717694262806,-0.848045003637552));
#134026=DIRECTION('ref_axis',(-3.7555222267109E-15,0.892442058026244,0.451162025292335));
#134027=DIRECTION('center_axis',(-0.809168721883308,0.587576360591314,-1.04314267264197E-13));
#134028=DIRECTION('ref_axis',(0.587576360591314,0.809168721883308,6.82961998416204E-15));
#134029=DIRECTION('center_axis',(0.587785252292496,0.809016994374931,-3.85528935811366E-14));
#134030=DIRECTION('ref_axis',(0.809016994374931,-0.587785252292496,-3.41480999208037E-15));
#134031=DIRECTION('center_axis',(-5.8046805746579E-17,-6.86903940691701E-15,
1.));
#134032=DIRECTION('ref_axis',(0.,-1.,-6.86903578052301E-15));
#134033=DIRECTION('center_axis',(-0.808865212939984,0.587994104813606,4.10594088861296E-15));
#134034=DIRECTION('ref_axis',(0.587994104813606,0.808865212939984,6.82961998416048E-15));
#134035=DIRECTION('center_axis',(0.587785252292471,0.809016994374949,5.73210557847752E-15));
#134036=DIRECTION('ref_axis',(0.809016994374949,-0.587785252292471,-3.41480999208039E-15));
#134037=DIRECTION('center_axis',(0.509008435041023,0.700641118228729,0.500012436349622));
#134038=DIRECTION('ref_axis',(-0.29470049257112,-0.403936649460554,0.866017784402214));
#134039=DIRECTION('center_axis',(-0.311481948263287,-0.428718122142695,
-0.848044673146732));
#134040=DIRECTION('ref_axis',(-4.34287574111871E-16,0.892441805934778,-0.451162523953256));
#134041=DIRECTION('center_axis',(-0.293895578893428,-0.40451254409655,-0.866022511471517));
#134042=DIRECTION('ref_axis',(-0.512651652661814,-0.697988741329765,0.500000000000001));
#134043=DIRECTION('center_axis',(0.293895578599952,0.404512560891358,0.866022503726384));
#134044=DIRECTION('ref_axis',(1.61736368199052E-15,-0.90603525611554,0.423202214875642));
#134045=DIRECTION('center_axis',(-0.311481949381041,-0.42871808065328,-0.848044693710629));
#134046=DIRECTION('ref_axis',(-0.502130522411202,-0.683410939228823,0.529919264233177));
#134047=DIRECTION('center_axis',(-0.311481909863924,-0.428718069290534,
-0.848044713969328));
#134048=DIRECTION('ref_axis',(-2.96332432358735E-15,0.892441837073399,-0.451162462358137));
#134049=DIRECTION('center_axis',(0.587785252292496,0.809016994374931,5.64933547733406E-15));
#134050=DIRECTION('ref_axis',(0.809016994374931,-0.587785252292496,-3.41480999208037E-15));
#134051=DIRECTION('center_axis',(-0.587785252292496,-0.809016994374931,
-5.64933547733406E-15));
#134052=DIRECTION('ref_axis',(-0.809016994374931,0.587785252292496,3.41480999208037E-15));
#134053=DIRECTION('center_axis',(0.587785252292471,0.809016994374949,5.73210557847752E-15));
#134054=DIRECTION('ref_axis',(0.809016994374949,-0.587785252292471,-3.41480999208039E-15));
#134055=DIRECTION('center_axis',(0.587785252292496,0.809016994374931,-5.85802630098928E-14));
#134056=DIRECTION('ref_axis',(0.809016994374931,-0.587785252292496,-3.41480999208036E-15));
#134057=DIRECTION('center_axis',(0.587785252292471,0.809016994374949,5.73210557847752E-15));
#134058=DIRECTION('ref_axis',(0.809016994374949,-0.587785252292471,-3.41480999208039E-15));
#134059=DIRECTION('center_axis',(-0.509016097474232,-0.700659176689747,
0.499979330205309));
#134060=DIRECTION('ref_axis',(-0.293100449224596,-0.405058175805674,-0.866036951219357));
#134061=DIRECTION('center_axis',(0.293895658256105,0.40451267052866,-0.866022425483303));
#134062=DIRECTION('ref_axis',(2.49577890397111E-15,0.906035197473505,0.423202340422576));
#134063=DIRECTION('center_axis',(0.293895663532304,0.40451267779073,-0.866022420300699));
#134064=DIRECTION('ref_axis',(-0.809016994372974,0.587785252295189,1.92322098297828E-12));
#134065=DIRECTION('center_axis',(-0.250002507179345,-0.433017044454286,
-0.866022508723715));
#134066=DIRECTION('ref_axis',(0.866025403784602,-0.499999999999718,-1.57354444798448E-13));
#134067=DIRECTION('center_axis',(-0.433035128830198,-0.749978760162002,
-0.500012436350217));
#134068=DIRECTION('ref_axis',(0.249149002240785,0.433518133164088,-0.866017784401882));
#134069=DIRECTION('center_axis',(0.250002511507192,0.433017051950262,0.866022503726318));
#134070=DIRECTION('ref_axis',(-4.36628801622752E-16,-0.894424794863792,
0.44721838774011));
#134071=DIRECTION('center_axis',(0.50000000000001,0.866025403784433,6.04742307255487E-15));
#134072=DIRECTION('ref_axis',(0.866025403784433,-0.50000000000001,-3.41480999208034E-15));
#134073=DIRECTION('center_axis',(-0.499999999999998,-0.86602540378444,-6.11783152599988E-15));
#134074=DIRECTION('ref_axis',(-0.86602540378444,0.499999999999998,3.41480999208033E-15));
#134075=DIRECTION('center_axis',(-0.50000000000001,-0.866025403784433,-6.04742307255487E-15));
#134076=DIRECTION('ref_axis',(-0.866025403784433,0.50000000000001,3.41480999208034E-15));
#134077=DIRECTION('center_axis',(-0.499999999999998,-0.86602540378444,-6.11783152599988E-15));
#134078=DIRECTION('ref_axis',(-0.86602540378444,0.499999999999998,3.41480999208033E-15));
#134079=DIRECTION('center_axis',(0.499999999999998,0.86602540378444,6.04742307255492E-15));
#134080=DIRECTION('ref_axis',(0.86602540378444,-0.499999999999998,-3.41480999208026E-15));
#134081=DIRECTION('center_axis',(-0.264962106632886,-0.458927830768635,
0.848045003637578));
#134082=DIRECTION('ref_axis',(1.98079904364529E-16,-0.879478602053326,-0.47593842934809));
#134083=DIRECTION('center_axis',(0.250002579266718,0.433017169313216,-0.866022425483289));
#134084=DIRECTION('ref_axis',(6.12936842783791E-16,0.894424730216417,0.447218517033106));
#134085=DIRECTION('center_axis',(0.264962073775778,0.458927817105223,-0.848045021297498));
#134086=DIRECTION('ref_axis',(0.420286434071742,0.736576463600215,0.529919264233205));
#134087=DIRECTION('center_axis',(-0.264962078570523,-0.458927782163196,
0.848045038708651));
#134088=DIRECTION('ref_axis',(-1.14611944484251E-15,-0.879478631391255,
-0.475938375135022));
#134089=DIRECTION('center_axis',(0.25000257708854,0.433017186565615,-0.866022417485764));
#134090=DIRECTION('ref_axis',(0.429067561974734,0.752263934574208,0.499999999999989));
#134091=DIRECTION('center_axis',(0.433048509462478,0.749993105181596,-0.499979330205153));
#134092=DIRECTION('ref_axis',(0.250824363776623,0.432512586705358,0.866036951219457));
#134093=DIRECTION('center_axis',(-0.866146626230631,0.499789977759954,3.49001476137941E-15));
#134094=DIRECTION('ref_axis',(0.499789977759954,0.866146626230631,6.82961998416062E-15));
#134095=DIRECTION('center_axis',(-0.499999999999998,-0.86602540378444,-6.11783152599988E-15));
#134096=DIRECTION('ref_axis',(-0.86602540378444,0.499999999999998,3.41480999208033E-15));
#134097=DIRECTION('center_axis',(0.500000000000051,0.866025403784409,6.04742307255471E-15));
#134098=DIRECTION('ref_axis',(0.866025403784409,-0.500000000000051,-3.41480999208024E-15));
#134099=DIRECTION('center_axis',(-7.04084534449556E-17,-6.86101165903726E-15,
1.));
#134100=DIRECTION('ref_axis',(0.,-1.,-6.86160339936723E-15));
#134101=DIRECTION('center_axis',(-0.865904130412286,0.500209992837952,3.49294771099313E-15));
#134102=DIRECTION('ref_axis',(0.500209992837952,0.865904130412285,6.82961998416082E-15));
#134103=DIRECTION('center_axis',(0.264962338412812,0.458928232223232,0.848044713969301));
#134104=DIRECTION('ref_axis',(-3.05791874716061E-15,-0.879478359737727,
0.47593887711873));
#134105=DIRECTION('center_axis',(0.264962078570518,0.458927782163202,-0.84804503870865));
#134106=DIRECTION('ref_axis',(1.10726528648156E-15,0.879478631391252,0.475938375135027));
#134107=DIRECTION('center_axis',(0.264962376554839,0.45892824786176,0.848044693589287));
#134108=DIRECTION('ref_axis',(-0.420092076161922,-0.736687329157012,0.529919264233218));
#134109=DIRECTION('center_axis',(0.264962371077221,0.458928288799647,0.848044673146743));
#134110=DIRECTION('ref_axis',(-4.96536252013644E-16,-0.879478325588514,
0.475938940222403));
#134111=DIRECTION('center_axis',(-0.264962073795953,-0.458927817276387,
0.848045021198568));
#134112=DIRECTION('ref_axis',(0.427750712262654,0.732266960577407,0.529919264233259));
#134113=DIRECTION('center_axis',(0.264962106632913,0.458927830768697,-0.848045003637535));
#134114=DIRECTION('ref_axis',(1.9774222481973E-15,0.879478602053289,0.475938429348159));
#134115=DIRECTION('center_axis',(-0.86615446498511,0.499776392786171,3.48991989801451E-15));
#134116=DIRECTION('ref_axis',(0.499776392786171,0.86615446498511,6.82961998416069E-15));
#134117=DIRECTION('center_axis',(0.50000000000001,0.866025403784433,-7.61181689576648E-15));
#134118=DIRECTION('ref_axis',(0.866025403784433,-0.50000000000001,-3.41480999208034E-15));
#134119=DIRECTION('center_axis',(-7.04084534449556E-17,-6.86101165903726E-15,
1.));
#134120=DIRECTION('ref_axis',(0.,-1.,-6.86152863759348E-15));
#134121=DIRECTION('center_axis',(-0.865896284857144,0.500223573885314,-1.6486202689183E-14));
#134122=DIRECTION('ref_axis',(0.500223573885314,0.865896284857144,6.8296199841604E-15));
#134123=DIRECTION('center_axis',(0.499999999999998,0.86602540378444,6.11783152599988E-15));
#134124=DIRECTION('ref_axis',(0.86602540378444,-0.499999999999998,-3.41480999208026E-15));
#134125=DIRECTION('center_axis',(0.432983094183966,0.750008802379043,0.500012436350171));
#134126=DIRECTION('ref_axis',(-0.250863215247218,-0.432528431823293,0.866017784401863));
#134127=DIRECTION('center_axis',(-0.264962371077247,-0.458928288799642,
-0.848044673146737));
#134128=DIRECTION('ref_axis',(7.54047727203941E-16,0.879478325588514,-0.475938940222403));
#134129=DIRECTION('center_axis',(-0.250002513555107,-0.433017035277681,
-0.86602251147153));
#134130=DIRECTION('ref_axis',(-0.436883602753634,-0.747751775420824,0.500000000000011));
#134131=DIRECTION('center_axis',(0.250002511507137,0.433017051950166,0.866022503726382));
#134132=DIRECTION('ref_axis',(-2.6848219789663E-16,-0.894424794863845,0.447218387740004));
#134133=DIRECTION('center_axis',(-0.264962376528037,-0.458928247653003,
-0.848044693710631));
#134134=DIRECTION('ref_axis',(-0.427943903632674,-0.732154074453082,0.529919264233127));
#134135=DIRECTION('center_axis',(-0.264962338412751,-0.458928232223233,
-0.848044713969319));
#134136=DIRECTION('ref_axis',(-3.1300340695229E-15,0.879478359737731,-0.475938877118722));
#134137=DIRECTION('center_axis',(0.50000000000001,0.866025403784433,-6.85880520999069E-14));
#134138=DIRECTION('ref_axis',(0.866025403784433,-0.50000000000001,-3.41480999208034E-15));
#134139=DIRECTION('center_axis',(-0.499999999999998,-0.86602540378444,-6.04742307255492E-15));
#134140=DIRECTION('ref_axis',(-0.86602540378444,0.499999999999998,3.41480999208026E-15));
#134141=DIRECTION('center_axis',(0.499999999999998,0.86602540378444,6.11783152599988E-15));
#134142=DIRECTION('ref_axis',(0.86602540378444,-0.499999999999998,-3.41480999208026E-15));
#134143=DIRECTION('center_axis',(0.50000000000001,0.866025403784433,-4.12695721632601E-14));
#134144=DIRECTION('ref_axis',(0.866025403784433,-0.50000000000001,-3.41480999208034E-15));
#134145=DIRECTION('center_axis',(0.499999999999998,0.86602540378444,6.11783152599988E-15));
#134146=DIRECTION('ref_axis',(0.86602540378444,-0.499999999999998,-3.41480999208026E-15));
#134147=DIRECTION('center_axis',(-0.432988827019191,-0.750027562856308,
0.499979330205132));
#134148=DIRECTION('ref_axis',(-0.249154705657247,-0.433476564270011,-0.866036951219471));
#134149=DIRECTION('center_axis',(0.250002579266723,0.433017169313225,-0.866022425483282));
#134150=DIRECTION('ref_axis',(2.19053741258821E-17,0.894424730216412,0.447218517033116));
#134151=DIRECTION('center_axis',(0.250002583755455,0.433017177087939,-0.866022420300069));
#134152=DIRECTION('ref_axis',(-0.86602540378426,0.500000000000309,2.22918795752825E-13));
#134153=DIRECTION('center_axis',(-0.203370361061543,-0.456777309666408,
-0.866022508723426));
#134154=DIRECTION('ref_axis',(0.913545457644901,-0.406736643070633,-3.26510472955345E-12));
#134155=DIRECTION('center_axis',(-0.35226878980237,-0.791134794599544,-0.500012436350449));
#134156=DIRECTION('ref_axis',(0.202469153687492,0.457186437796381,-0.866017784401756));
#134157=DIRECTION('center_axis',(0.203370364581923,0.456777317573264,0.866022503726311));
#134158=DIRECTION('ref_axis',(-1.56869163259611E-15,-0.884507036382102,
0.466526850878436));
#134159=DIRECTION('center_axis',(0.406736643075797,0.913545457642603,6.37925383508811E-15));
#134160=DIRECTION('ref_axis',(0.913545457642603,-0.406736643075797,-3.41480999208023E-15));
#134161=DIRECTION('center_axis',(-0.406736643075798,-0.913545457642602,
-6.43652923108483E-15));
#134162=DIRECTION('ref_axis',(-0.913545457642602,0.406736643075798,3.41480999208033E-15));
#134163=DIRECTION('center_axis',(-0.406736643075807,-0.913545457642598,
-6.37925383508808E-15));
#134164=DIRECTION('ref_axis',(-0.913545457642598,0.406736643075807,3.4148099920803E-15));
#134165=DIRECTION('center_axis',(-0.406736643075798,-0.913545457642602,
-6.43652923108483E-15));
#134166=DIRECTION('ref_axis',(-0.913545457642602,0.406736643075798,3.41480999208033E-15));
#134167=DIRECTION('center_axis',(0.406736643075817,0.913545457642594,6.37925383508805E-15));
#134168=DIRECTION('ref_axis',(0.913545457642593,-0.406736643075817,-3.41480999208037E-15));
#134169=DIRECTION('center_axis',(-0.215539595588311,-0.484109857923786,
0.848045003637566));
#134170=DIRECTION('ref_axis',(1.22794633366769E-15,-0.868458021515985,-0.495762710240031));
#134171=DIRECTION('center_axis',(0.203370419702463,0.456777441376078,-0.866022425483294));
#134172=DIRECTION('ref_axis',(-1.81222983169436E-15,0.884506966812057,0.466526982779062));
#134173=DIRECTION('center_axis',(0.21553956433415,0.484109840903014,-0.848045021297516));
#134174=DIRECTION('ref_axis',(0.340990855172982,0.776473315757201,0.529919264233163));
#134175=DIRECTION('center_axis',(-0.215539572760312,-0.48410980665126,0.848045038708666));
#134176=DIRECTION('ref_axis',(-2.44700238975538E-15,-0.868458052949974,
-0.495762655175175));
#134177=DIRECTION('center_axis',(0.203370415728145,0.456777458308414,-0.866022417485752));
#134178=DIRECTION('ref_axis',(0.348084091910994,0.792992726926611,0.499999999999996));
#134179=DIRECTION('center_axis',(0.352280597671115,0.791150459692777,-0.499979330205149));
#134180=DIRECTION('ref_axis',(0.204240445631702,0.456361522798167,0.866036951219463));
#134181=DIRECTION('center_axis',(-0.913644062717548,0.406515100163541,2.8386797723579E-15));
#134182=DIRECTION('ref_axis',(0.406515100163541,0.913644062717548,6.82961998416062E-15));
#134183=DIRECTION('center_axis',(-0.406736643075798,-0.913545457642602,
-6.43652923108483E-15));
#134184=DIRECTION('ref_axis',(-0.913545457642602,0.406736643075798,3.41480999208033E-15));
#134185=DIRECTION('center_axis',(0.406736643075807,0.913545457642598,6.37925383508808E-15));
#134186=DIRECTION('ref_axis',(0.913545457642598,-0.406736643075807,-3.4148099920803E-15));
#134187=DIRECTION('center_axis',(-8.35415108931911E-17,-6.85432003203771E-15,
1.));
#134188=DIRECTION('ref_axis',(0.,-1.,-6.85455139176254E-15));
#134189=DIRECTION('center_axis',(-0.913446798847332,0.406958162070208,2.84177365711606E-15));
#134190=DIRECTION('ref_axis',(0.406958162070208,0.913446798847332,6.82961998416058E-15));
#134191=DIRECTION('center_axis',(0.215539784135028,0.484110281406733,0.848044713969328));
#134192=DIRECTION('ref_axis',(-1.26159198727182E-15,-0.86845776188828,0.495763165045568));
#134193=DIRECTION('center_axis',(0.215539572760318,0.484109806651275,-0.848045038708655));
#134194=DIRECTION('ref_axis',(1.56117104191503E-15,0.868458052949965,0.495762655175191));
#134195=DIRECTION('center_axis',(0.215539820433354,0.484110300946589,0.848044693589295));
#134196=DIRECTION('ref_axis',(-0.340785973376786,-0.776563258044201,0.529919264233158));
#134197=DIRECTION('center_axis',(0.215539810706706,0.4841103410876,0.848044673146743));
#134198=DIRECTION('ref_axis',(-1.47259052727932E-15,-0.868457725299275,
0.495763229140694));
#134199=DIRECTION('center_axis',(-0.215539564338139,-0.484109841074578,
0.848045021198564));
#134200=DIRECTION('ref_axis',(0.348864709021599,0.772967650159955,0.529919264233216));
#134201=DIRECTION('center_axis',(0.215539595588311,0.484109857923786,-0.848045003637566));
#134202=DIRECTION('ref_axis',(-1.22794633366769E-15,0.868458021515985,0.495762710240031));
#134203=DIRECTION('center_axis',(-0.913650438514067,0.406500770236727,2.7798120880666E-14));
#134204=DIRECTION('ref_axis',(0.406500770236727,0.913650438514067,6.82961998416101E-15));
#134205=DIRECTION('center_axis',(0.406736643075807,0.913545457642598,6.37925383508808E-15));
#134206=DIRECTION('ref_axis',(0.913545457642598,-0.406736643075807,-3.4148099920803E-15));
#134207=DIRECTION('center_axis',(-8.35415108931911E-17,-6.85432003203771E-15,
1.));
#134208=DIRECTION('ref_axis',(0.,-1.,-6.85402149466395E-15));
#134209=DIRECTION('center_axis',(-0.913440415876952,0.406972488803039,1.23809565966439E-16));
#134210=DIRECTION('ref_axis',(0.406972488803039,0.913440415876953,6.82961998416061E-15));
#134211=DIRECTION('center_axis',(0.406736643075798,0.913545457642602,6.43652923108483E-15));
#134212=DIRECTION('ref_axis',(0.913545457642602,-0.406736643075798,-3.41480999208024E-15));
#134213=DIRECTION('center_axis',(0.352213899942024,0.791159233141463,0.500012436347979));
#134214=DIRECTION('ref_axis',(-0.204277427918833,-0.456381342234996,0.866017784403213));
#134215=DIRECTION('center_axis',(-0.215539810706709,-0.484110341087593,
-0.848044673146745));
#134216=DIRECTION('ref_axis',(1.74357575843794E-15,0.868457725299279,-0.495763229140688));
#134217=DIRECTION('center_axis',(-0.203370368360526,-0.456777301206467,
-0.866022511471521));
#134218=DIRECTION('ref_axis',(-0.356328964673919,-0.789322284579871,0.500000000000026));
#134219=DIRECTION('center_axis',(0.203370364581877,0.456777317573187,0.866022503726363));
#134220=DIRECTION('ref_axis',(-7.57999114950329E-16,-0.884507036382146,
0.466526850878353));
#134221=DIRECTION('center_axis',(-0.215539820428636,-0.484110300736156,
-0.84804469371062));
#134222=DIRECTION('ref_axis',(-0.349068641879027,-0.772875576436027,0.529919264233156));
#134223=DIRECTION('center_axis',(-0.21553978413504,-0.484110281406725,-0.84804471396933));
#134224=DIRECTION('ref_axis',(1.68002389095411E-15,0.868457761888284,-0.495763165045561));
#134225=DIRECTION('center_axis',(0.406736643075807,0.913545457642598,6.37925383508808E-15));
#134226=DIRECTION('ref_axis',(0.913545457642598,-0.406736643075807,-3.4148099920803E-15));
#134227=DIRECTION('center_axis',(-0.406736643075797,-0.913545457642603,
-6.37925383508811E-15));
#134228=DIRECTION('ref_axis',(-0.913545457642603,0.406736643075797,3.41480999208023E-15));
#134229=DIRECTION('center_axis',(0.406736643075798,0.913545457642602,6.43652923108483E-15));
#134230=DIRECTION('ref_axis',(0.913545457642602,-0.406736643075798,-3.41480999208024E-15));
#134231=DIRECTION('center_axis',(0.406736643075807,0.913545457642598,-4.35340926765517E-14));
#134232=DIRECTION('ref_axis',(0.913545457642598,-0.406736643075807,-3.4148099920803E-15));
#134233=DIRECTION('center_axis',(0.406736643075798,0.913545457642602,6.43652923108483E-15));
#134234=DIRECTION('ref_axis',(0.913545457642602,-0.406736643075798,-3.41480999208024E-15));
#134235=DIRECTION('center_axis',(-0.352217640366521,-0.791178490090796,
0.499979330205049));
#134236=DIRECTION('ref_axis',(-0.202479170981813,-0.457145692794892,-0.866036951219517));
#134237=DIRECTION('center_axis',(0.20337041970247,0.456777441376081,-0.866022425483291));
#134238=DIRECTION('ref_axis',(-2.00922857707489E-15,0.884506966812055,0.466526982779065));
#134239=DIRECTION('center_axis',(0.203370423351993,0.456777449573005,-0.866022420302853));
#134240=DIRECTION('ref_axis',(-0.91354545764246,0.406736643076116,1.61725400840202E-13));
#134241=DIRECTION('center_axis',(-0.154510046710251,-0.475533027088399,
-0.866022508722343));
#134242=DIRECTION('ref_axis',(0.951056516294649,-0.309016994376501,9.57239539185634E-13));
#134243=DIRECTION('center_axis',(-0.267642920194609,-0.823622990673633,
-0.50001243634886));
#134244=DIRECTION('ref_axis',(0.153571010704088,0.475845712147976,-0.866017784402671));
#134245=DIRECTION('center_axis',(0.154510049384272,0.475533035318147,0.866022503726306));
#134246=DIRECTION('ref_axis',(1.85643597775053E-15,-0.876548788012432,0.481313018974073));
#134247=DIRECTION('center_axis',(0.309016994374956,0.951056516295151,5.86040288757031E-14));
#134248=DIRECTION('ref_axis',(0.951056516295151,-0.309016994374956,-3.41480999207978E-15));
#134249=DIRECTION('center_axis',(-0.309016994374945,-0.951056516295154,
-6.68470697498368E-15));
#134250=DIRECTION('ref_axis',(-0.951056516295154,0.309016994374945,3.41480999208033E-15));
#134251=DIRECTION('center_axis',(-0.309016994374964,-0.951056516295148,
-5.01621543147891E-14));
#134252=DIRECTION('ref_axis',(-0.951056516295148,0.309016994374964,3.41480999207994E-15));
#134253=DIRECTION('center_axis',(-0.309016994374945,-0.951056516295154,
-6.68470697498368E-15));
#134254=DIRECTION('ref_axis',(-0.951056516295154,0.309016994374945,3.41480999208033E-15));
#134255=DIRECTION('center_axis',(0.309016994374972,0.951056516295146,6.64119215765932E-15));
#134256=DIRECTION('ref_axis',(0.951056516295146,-0.309016994374972,-3.41480999208037E-15));
#134257=DIRECTION('center_axis',(-0.163755587629913,-0.50398787616902,0.848045003637556));
#134258=DIRECTION('ref_axis',(1.74588362472744E-15,-0.859649462041466,-0.510884333691901));
#134259=DIRECTION('center_axis',(0.154510091261934,0.475533164204418,-0.866022425483291));
#134260=DIRECTION('ref_axis',(-8.93385339497672E-16,0.876548714628834,0.48131315261744));
#134261=DIRECTION('center_axis',(0.163755558326672,0.503987855974368,-0.848045021297501));
#134262=DIRECTION('ref_axis',(0.257959309137026,0.807862963765574,0.529919264233195));
#134263=DIRECTION('center_axis',(-0.16375557028641,-0.503987822791206,0.848045038708648));
#134264=DIRECTION('ref_axis',(-1.88791329792594E-15,-0.859649495083702,
-0.510884278092736));
#134265=DIRECTION('center_axis',(0.154510085545305,0.47553318062662,-0.866022417485779));
#134266=DIRECTION('ref_axis',(0.263286939716706,0.825033325008545,0.499999999999957));
#134267=DIRECTION('center_axis',(0.26765302593241,0.82363980420871,-0.499979330205022));
#134268=DIRECTION('ref_axis',(0.155418826426913,0.475210466545561,0.866036951219537));
#134269=DIRECTION('center_axis',(-0.951131423661017,0.308786358060986,2.15624361371854E-15));
#134270=DIRECTION('ref_axis',(0.308786358060986,0.951131423661017,6.82961998416067E-15));
#134271=DIRECTION('center_axis',(-0.309016994374945,-0.951056516295154,
-6.68470697498368E-15));
#134272=DIRECTION('ref_axis',(-0.951056516295154,0.309016994374945,3.41480999208033E-15));
#134273=DIRECTION('center_axis',(0.309016994374922,0.951056516295162,6.64119215765944E-15));
#134274=DIRECTION('ref_axis',(0.951056516295162,-0.309016994374922,-3.41480999208039E-15));
#134275=DIRECTION('center_axis',(-9.73020895656139E-17,-6.84903784078409E-15,
1.));
#134276=DIRECTION('ref_axis',(0.,-1.,-6.84749938415785E-15));
#134277=DIRECTION('center_axis',(-0.95098155300316,0.309247612517378,2.15946453637244E-15));
#134278=DIRECTION('ref_axis',(0.309247612517378,0.95098155300316,6.82961998416082E-15));
#134279=DIRECTION('center_axis',(0.163755730877736,0.503988317040564,0.848044713969328));
#134280=DIRECTION('ref_axis',(1.3688970201719E-17,-0.859649189130477,0.510884792910607));
#134281=DIRECTION('center_axis',(0.163755570286409,0.503987822791204,-0.84804503870865));
#134282=DIRECTION('ref_axis',(1.78266007267482E-15,0.859649495083703,0.510884278092735));
#134283=DIRECTION('center_axis',(0.16375576493453,0.503988340267678,0.848044693589281));
#134284=DIRECTION('ref_axis',(-0.257746148173953,-0.807930997360561,0.529919264233203));
#134285=DIRECTION('center_axis',(0.163755751065515,0.503988379171995,0.848044673146736));
#134286=DIRECTION('ref_axis',(-2.42242054595195E-15,-0.859649150669468,
0.510884857627686));
#134287=DIRECTION('center_axis',(-0.163755558317466,-0.50398785614383,0.848045021198569));
#134288=DIRECTION('ref_axis',(0.26615647101259,0.805199544419036,0.529919264233243));
#134289=DIRECTION('center_axis',(0.1637555876299,0.50398787616898,-0.848045003637583));
#134290=DIRECTION('ref_axis',(4.71498135796894E-16,0.859649462041491,0.510884333691859));
#134291=DIRECTION('center_axis',(-0.951136266645027,0.308771440182801,-6.95712478733955E-15));
#134292=DIRECTION('ref_axis',(0.308771440182801,0.951136266645027,6.82961998416065E-15));
#134293=DIRECTION('center_axis',(0.309016994374964,0.951056516295148,-4.53216445603843E-14));
#134294=DIRECTION('ref_axis',(0.951056516295148,-0.309016994374964,-3.41480999208075E-15));
#134295=DIRECTION('center_axis',(-9.73020895656139E-17,-6.84903784078409E-15,
1.));
#134296=DIRECTION('ref_axis',(0.,-1.,-6.84651435173441E-15));
#134297=DIRECTION('center_axis',(-0.950976702550722,0.309262527968967,-6.92250494748091E-15));
#134298=DIRECTION('ref_axis',(0.309262527968967,0.950976702550722,6.8296199841605E-15));
#134299=DIRECTION('center_axis',(0.309016994374945,0.951056516295154,6.68470697498368E-15));
#134300=DIRECTION('ref_axis',(0.951056516295154,-0.309016994374945,-3.41480999208036E-15));
#134301=DIRECTION('center_axis',(0.267585776505841,0.823641557783774,0.500012436348622));
#134302=DIRECTION('ref_axis',(-0.155453534525656,-0.475234043079439,0.866017784402751));
#134303=DIRECTION('center_axis',(-0.163755751065466,-0.503988379171994,
-0.848044673146746));
#134304=DIRECTION('ref_axis',(-1.95984699059842E-15,0.859649150669472,-0.51088485762768));
#134305=DIRECTION('center_axis',(-0.154510054857039,-0.475533019434617,
-0.866022511471539));
#134306=DIRECTION('ref_axis',(-0.27187031189046,-0.822244813612451,0.50000000000001));
#134307=DIRECTION('center_axis',(0.154510049384245,0.475533035317994,0.866022503726395));
#134308=DIRECTION('ref_axis',(-3.62116518657123E-16,-0.876548788012518,
0.481313018973917));
#134309=DIRECTION('center_axis',(-0.163755764949564,-0.503988340058636,
-0.848044693710611));
#134310=DIRECTION('ref_axis',(-0.266368911015363,-0.805129291877427,0.529919264233188));
#134311=DIRECTION('center_axis',(-0.16375573087769,-0.503988317040571,-0.848044713969332));
#134312=DIRECTION('ref_axis',(3.12513560129423E-16,0.859649189130475,-0.51088479291061));
#134313=DIRECTION('center_axis',(0.309016994374964,0.951056516295148,1.50830667185733E-14));
#134314=DIRECTION('ref_axis',(0.951056516295148,-0.309016994374964,-3.41480999208024E-15));
#134315=DIRECTION('center_axis',(-0.309016994374964,-0.951056516295148,
-6.64119215765934E-15));
#134316=DIRECTION('ref_axis',(-0.951056516295148,0.309016994374964,3.41480999208031E-15));
#134317=DIRECTION('center_axis',(0.309016994374945,0.951056516295154,6.68470697498368E-15));
#134318=DIRECTION('ref_axis',(0.951056516295154,-0.309016994374945,-3.41480999208036E-15));
#134319=DIRECTION('center_axis',(0.309016994374964,0.951056516295148,-6.22053936822121E-14));
#134320=DIRECTION('ref_axis',(0.951056516295148,-0.309016994374964,-3.41480999208089E-15));
#134321=DIRECTION('center_axis',(0.309016994374945,0.951056516295154,6.68470697498368E-15));
#134322=DIRECTION('ref_axis',(0.951056516295154,-0.309016994374945,-3.41480999208036E-15));
#134323=DIRECTION('center_axis',(-0.267587483540256,-0.82366110022265,0.499979330205367));
#134324=DIRECTION('ref_axis',(-0.15358523212817,-0.475806237448477,-0.866036951219323));
#134325=DIRECTION('center_axis',(0.154510091261981,0.475533164204423,-0.86602242548328));
#134326=DIRECTION('ref_axis',(-1.07558166235271E-15,0.876548714628829,0.481313152617449));
#134327=DIRECTION('center_axis',(0.154510094033318,0.475533172733701,-0.866022420305407));
#134328=DIRECTION('ref_axis',(-0.951056516296803,0.309016994369873,-3.0946373998982E-12));
#134329=DIRECTION('center_axis',(-0.10395688795453,-0.489078705158565,-0.866022508718584));
#134330=DIRECTION('ref_axis',(0.978147600733646,-0.207911690818511,4.5895046399331E-13));
#134331=DIRECTION('center_axis',(-0.180084698746432,-0.847087400906293,
-0.500012436348566));
#134332=DIRECTION('ref_axis',(0.102990311619474,0.489291521294292,-0.866017784402861));
#134333=DIRECTION('center_axis',(0.103956889752271,0.489078713616363,0.866022503726317));
#134334=DIRECTION('ref_axis',(-3.34623636700672E-16,-0.870740345484707,
0.49174307391683));
#134335=DIRECTION('center_axis',(0.20791169081776,0.978147600733806,-4.66126430222498E-14));
#134336=DIRECTION('ref_axis',(0.978147600733806,-0.20791169081776,1.32038128099746E-28));
#134337=DIRECTION('center_axis',(-0.207911690817756,-0.978147600733806,
-6.85964567039975E-15));
#134338=DIRECTION('ref_axis',(-0.978147600733806,0.207911690817756,4.65131225051149E-31));
#134339=DIRECTION('center_axis',(-0.207911690817757,-0.978147600733806,
-6.83036818919254E-15));
#134340=DIRECTION('ref_axis',(-0.978147600733806,0.207911690817757,-2.9624920046404E-32));
#134341=DIRECTION('center_axis',(-0.207911690817756,-0.978147600733806,
-6.85964567039975E-15));
#134342=DIRECTION('ref_axis',(-0.978147600733806,0.207911690817756,-4.9939677714214E-31));
#134343=DIRECTION('center_axis',(0.207911690817754,0.978147600733807,6.83036818919254E-15));
#134344=DIRECTION('ref_axis',(0.978147600733807,-0.207911690817754,1.95800148050649E-29));
#134345=DIRECTION('center_axis',(-0.110177439185354,-0.518344097776659,
0.848045003637578));
#134346=DIRECTION('ref_axis',(-1.54555453578699E-15,-0.853239582811865,
-0.521519140898045));
#134347=DIRECTION('center_axis',(0.103956917928293,0.489078846174045,-0.866022425483264));
#134348=DIRECTION('ref_axis',(-1.23054211610355E-15,0.870740269393752,0.491743208652745));
#134349=DIRECTION('center_axis',(0.110177412156739,0.518344074628991,-0.848045021297489));
#134350=DIRECTION('ref_axis',(0.172101506937256,0.830401496087534,0.529919264233252));
#134351=DIRECTION('center_axis',(-0.110177427516371,-0.518344042878412,
0.848045038708639));
#134352=DIRECTION('ref_axis',(8.08042342219762E-16,-0.853239616987295,-0.521519084984792));
#134353=DIRECTION('center_axis',(0.103956910525269,0.48907886190895,-0.866022417485764));
#134354=DIRECTION('ref_axis',(0.175605160703735,0.848034685336757,0.500000000000003));
#134355=DIRECTION('center_axis',(0.180092991630818,0.847105178672015,-0.499979330205275));
#134356=DIRECTION('ref_axis',(0.104894406050269,0.488852904974495,0.86603695121938));
#134357=DIRECTION('center_axis',(-0.978197989689806,0.20767448800183,1.45018319882439E-15));
#134358=DIRECTION('ref_axis',(0.20767448800183,0.978197989689806,6.82961998416083E-15));
#134359=DIRECTION('center_axis',(-0.207911690817756,-0.978147600733806,
-6.85964567039975E-15));
#134360=DIRECTION('ref_axis',(-0.978147600733806,0.207911690817756,4.65131225051149E-31));
#134361=DIRECTION('center_axis',(0.207911690817757,0.978147600733806,6.83036818919254E-15));
#134362=DIRECTION('ref_axis',(0.978147600733806,-0.207911690817757,2.9624920046404E-32));
#134363=DIRECTION('center_axis',(-1.11539425682703E-16,-6.84522295806915E-15,
1.));
#134364=DIRECTION('ref_axis',(0.,-1.,-6.84749938415785E-15));
#134365=DIRECTION('center_axis',(-0.978097154258596,0.208148881407602,1.45349587027143E-15));
#134366=DIRECTION('ref_axis',(0.208148881407602,0.978097154258596,6.82961998416047E-15));
#134367=DIRECTION('center_axis',(0.110177535564839,0.518344551206562,0.848044713969333));
#134368=DIRECTION('ref_axis',(1.17513314922421E-15,-0.853239300541054,0.521519602711358));
#134369=DIRECTION('center_axis',(0.110177427516339,0.518344042878482,-0.848045038708601));
#134370=DIRECTION('ref_axis',(-1.26528534754762E-16,0.853239616987253,0.521519084984861));
#134371=DIRECTION('center_axis',(0.110177567011267,0.518344577865476,0.848044693589282));
#134372=DIRECTION('ref_axis',(-0.171882402210563,-0.830446875606688,0.529919264233162));
#134373=DIRECTION('center_axis',(0.110177549147492,0.518344615107833,0.848044673146742));
#134374=DIRECTION('ref_axis',(1.16486514661486E-15,-0.853239260760976,0.521519667794095));
#134375=DIRECTION('center_axis',(-0.110177412123957,-0.518344074797815,
0.84804502119856));
#134376=DIRECTION('ref_axis',(0.1805321670207,0.828609503967533,0.529919264233231));
#134377=DIRECTION('center_axis',(0.110177439185352,0.51834409777665,-0.848045003637584));
#134378=DIRECTION('ref_axis',(-1.32803749140163E-15,0.853239582811871,0.521519140898035));
#134379=DIRECTION('center_axis',(-0.978201246800567,0.207659145615639,-5.65545097523496E-16));
#134380=DIRECTION('ref_axis',(0.207659145615639,0.978201246800567,6.82961998416065E-15));
#134381=DIRECTION('center_axis',(0.207911690817757,0.978147600733806,6.83036818919254E-15));
#134382=DIRECTION('ref_axis',(0.978147600733806,-0.207911690817757,2.9624920046404E-32));
#134383=DIRECTION('center_axis',(-1.11539425682703E-16,-6.84522295806915E-15,
1.));
#134384=DIRECTION('ref_axis',(0.,-1.,-6.84651435173441E-15));
#134385=DIRECTION('center_axis',(-0.978093889466682,0.208164222161104,1.45360299418058E-15));
#134386=DIRECTION('ref_axis',(0.208164222161104,0.978093889466682,6.82961998416055E-15));
#134387=DIRECTION('center_axis',(0.207911690817756,0.978147600733806,6.85964567039975E-15));
#134388=DIRECTION('ref_axis',(0.978147600733806,-0.207911690817756,-5.48498646232285E-30));
#134389=DIRECTION('center_axis',(0.180025927304963,0.847099893161503,0.500012436349096));
#134390=DIRECTION('ref_axis',(-0.104926459548316,-0.488879980348169,0.866017784402509));
#134391=DIRECTION('center_axis',(-0.110177549147462,-0.518344615107834,
-0.848044673146745));
#134392=DIRECTION('ref_axis',(-1.35828912679475E-15,0.853239260760977,-0.521519667794094));
#134393=DIRECTION('center_axis',(-0.103956896854893,-0.489078698392047,
-0.866022511471522));
#134394=DIRECTION('ref_axis',(-0.184432991087763,-0.846158656398667,0.500000000000023));
#134395=DIRECTION('center_axis',(0.103956889752284,0.489078713616327,0.866022503726335));
#134396=DIRECTION('ref_axis',(-1.08655637743655E-15,-0.870740345484727,
0.491743073916795));
#134397=DIRECTION('center_axis',(-0.110177567046589,-0.518344577659445,
-0.848044693710624));
#134398=DIRECTION('ref_axis',(-0.180750786634256,-0.828561842306085,0.529919264233189));
#134399=DIRECTION('center_axis',(-0.110177535564859,-0.518344551206569,
-0.848044713969325));
#134400=DIRECTION('ref_axis',(1.46521819382421E-15,0.853239300541049,-0.521519602711367));
#134401=DIRECTION('center_axis',(0.207911690817757,0.978147600733806,6.83036818919254E-15));
#134402=DIRECTION('ref_axis',(0.978147600733806,-0.207911690817757,2.9624920046404E-32));
#134403=DIRECTION('center_axis',(-0.207911690817754,-0.978147600733807,
-6.83036818919254E-15));
#134404=DIRECTION('ref_axis',(-0.978147600733807,0.207911690817754,-1.95800148050649E-29));
#134405=DIRECTION('center_axis',(0.207911690817756,0.978147600733806,6.85964567039975E-15));
#134406=DIRECTION('ref_axis',(0.978147600733806,-0.207911690817756,-5.48498646232285E-30));
#134407=DIRECTION('center_axis',(0.207911690817757,0.978147600733806,-1.68937884210484E-15));
#134408=DIRECTION('ref_axis',(0.978147600733806,-0.207911690817757,4.04710180979884E-32));
#134409=DIRECTION('center_axis',(0.207911690817756,0.978147600733806,6.85964567039975E-15));
#134410=DIRECTION('ref_axis',(0.978147600733806,-0.207911690817756,-5.48498646232285E-30));
#134411=DIRECTION('center_axis',(-0.180025582247582,-0.847119506978666,
0.499979330205401));
#134412=DIRECTION('ref_axis',(-0.103008581356496,-0.489253749387449,-0.866036951219315));
#134413=DIRECTION('center_axis',(0.103956917928286,0.489078846174007,-0.866022425483286));
#134414=DIRECTION('ref_axis',(-1.08851636843951E-16,0.870740269393773,0.491743208652707));
#134415=DIRECTION('center_axis',(0.103956919794677,0.489078854954631,-0.866022420300462));
#134416=DIRECTION('ref_axis',(-0.978147600734682,0.207911690813636,-2.45647771009641E-12));
#134417=DIRECTION('center_axis',(-0.0522647557773232,-0.497265934576513,
-0.866022508722079));
#134418=DIRECTION('ref_axis',(0.994521895368419,-0.104528463266268,-7.73659353600025E-13));
#134419=DIRECTION('center_axis',(-0.0905534316550513,-0.861270944309439,
-0.500012436349159));
#134420=DIRECTION('ref_axis',(0.051281229102223,0.497376550151214,-0.866017784402516));
#134421=DIRECTION('center_axis',(0.0522647566818157,0.497265943181911,0.866022503726315));
#134422=DIRECTION('ref_axis',(5.43068232277855E-16,-0.867207748104381,0.497946504785131));
#134423=DIRECTION('center_axis',(0.104528463267629,0.994521895368276,6.94470927749848E-15));
#134424=DIRECTION('ref_axis',(0.994521895368276,-0.104528463267629,-4.99922698313062E-30));
#134425=DIRECTION('center_axis',(-0.10452846326765,-0.994521895368274,-6.95942865237777E-15));
#134426=DIRECTION('ref_axis',(-0.994521895368274,0.10452846326765,-1.06118964965575E-32));
#134427=DIRECTION('center_axis',(-0.104528463267629,-0.994521895368276,
-6.23081959585229E-15));
#134428=DIRECTION('ref_axis',(-0.994521895368276,0.104528463267629,4.55502821820944E-30));
#134429=DIRECTION('center_axis',(-0.10452846326765,-0.994521895368274,-6.95942865237777E-15));
#134430=DIRECTION('ref_axis',(-0.994521895368274,0.10452846326765,-1.06118964965575E-32));
#134431=DIRECTION('center_axis',(0.104528463267629,0.994521895368276,6.94470927749848E-15));
#134432=DIRECTION('ref_axis',(0.994521895368276,-0.104528463267629,-4.99922698313062E-30));
#134433=DIRECTION('center_axis',(-0.0553921636609753,-0.527021232978594,
0.848045003637589));
#134434=DIRECTION('ref_axis',(3.12484149181909E-16,-0.84934903001939,-0.5278316258099));
#134435=DIRECTION('center_axis',(0.0522647708473854,0.497266077958579,-0.866022425483291));
#134436=DIRECTION('ref_axis',(-1.07267863460433E-16,0.867207670398078,0.497946640115924));
#134437=DIRECTION('center_axis',(0.0553921391963296,0.527021207132855,-0.848045021297503));
#134438=DIRECTION('ref_axis',(0.0843581245585095,0.843841975855393,0.529919264233182));
#134439=DIRECTION('center_axis',(-0.0553921577943468,-0.527021177161352,
0.848045038708646));
#134440=DIRECTION('ref_axis',(-2.92497129473667E-16,-0.849349064867516,
-0.527831569734774));
#134441=DIRECTION('center_axis',(0.0522647618413962,0.497266092833347,-0.866022417485783));
#134442=DIRECTION('ref_axis',(0.0859994148076584,0.861744800189005,0.499999999999952));
#134443=DIRECTION('center_axis',(0.0905598208271191,0.861289491529708,-0.499979330205016));
#134444=DIRECTION('ref_axis',(0.0532207405910698,0.497139368681772,0.866036951219535));
#134445=DIRECTION('center_axis',(-0.994547213842469,0.104287292793432,-6.06414525351624E-15));
#134446=DIRECTION('ref_axis',(0.104287292793432,0.994547213842469,6.82961998416055E-15));
#134447=DIRECTION('center_axis',(-0.10452846326765,-0.994521895368274,-6.95942865237777E-15));
#134448=DIRECTION('ref_axis',(-0.994521895368274,0.10452846326765,-1.06118964965575E-32));
#134449=DIRECTION('center_axis',(0.104528463267628,0.994521895368276,6.94470927749848E-15));
#134450=DIRECTION('ref_axis',(0.994521895368276,-0.104528463267628,1.09814391166396E-31));
#134451=DIRECTION('center_axis',(-1.26097532010604E-16,-6.84291718054622E-15,
1.));
#134452=DIRECTION('ref_axis',(0.,-1.,-6.84044737655315E-15));
#134453=DIRECTION('center_axis',(-0.994496518411991,0.10476962759516,7.3160239925209E-16));
#134454=DIRECTION('ref_axis',(0.10476962759516,0.994496518411991,6.82961998416045E-15));
#134455=DIRECTION('center_axis',(0.0553922121161709,0.527021693998976,0.848044713969333));
#134456=DIRECTION('ref_axis',(7.77180288600867E-16,-0.849348742192416,0.527832088960269));
#134457=DIRECTION('center_axis',(0.0553921577943474,0.527021177161358,-0.848045038708643));
#134458=DIRECTION('ref_axis',(8.49466062352983E-17,0.849349064867513,0.52783156973478));
#134459=DIRECTION('center_axis',(0.0553922406021807,0.527021723799047,0.848044693589289));
#134460=DIRECTION('ref_axis',(-0.0841354766906324,-0.843864204097235,0.529919264233128));
#134461=DIRECTION('center_axis',(0.0553922189448978,0.527021758969969,0.84804467314674));
#134462=DIRECTION('ref_axis',(-1.4399498926774E-16,-0.849348701629312,0.527832154231438));
#134463=DIRECTION('center_axis',(-0.0553921391403666,-0.527021207297975,
0.848045021198544));
#134464=DIRECTION('ref_axis',(0.0929299148375028,0.842941044393284,0.529919264233197));
#134465=DIRECTION('center_axis',(0.0553921636609804,0.527021232978642,-0.848045003637559));
#134466=DIRECTION('ref_axis',(3.75742388398108E-16,0.849349030019359,0.527831625809948));
#134467=DIRECTION('center_axis',(-0.994548849394383,0.104271693993668,7.28125347496908E-16));
#134468=DIRECTION('ref_axis',(0.104271693993668,0.994548849394383,6.8296199841608E-15));
#134469=DIRECTION('center_axis',(0.104528463267629,0.994521895368276,6.23081959585229E-15));
#134470=DIRECTION('ref_axis',(0.994521895368276,-0.104528463267629,-4.55502821820944E-30));
#134471=DIRECTION('center_axis',(-1.26097532010604E-16,-6.84291718054622E-15,
1.));
#134472=DIRECTION('ref_axis',(0.,-1.,-6.84651435173441E-15));
#134473=DIRECTION('center_axis',(-0.994494875050338,0.104785225574086,6.45685748436114E-15));
#134474=DIRECTION('ref_axis',(0.104785225574086,0.994494875050338,6.82961998416065E-15));
#134475=DIRECTION('center_axis',(0.10452846326765,0.994521895368274,6.95942865237777E-15));
#134476=DIRECTION('ref_axis',(0.994521895368274,-0.10452846326765,-8.52179472506115E-30));
#134477=DIRECTION('center_axis',(0.0904936763725661,0.86127722484297,0.500012436348706));
#134478=DIRECTION('ref_axis',(-0.0532497883514946,-0.497169646236267,0.866017784402737));
#134479=DIRECTION('center_axis',(-0.0553922189448982,-0.527021758969977,
-0.848044673146735));
#134480=DIRECTION('ref_axis',(1.29981789962805E-16,0.849348701629308,-0.527832154231446));
#134481=DIRECTION('center_axis',(-0.0522647653362515,-0.497265928783454,
-0.866022511471541));
#134482=DIRECTION('ref_axis',(-0.0949749838229919,-0.860801807879048,0.499999999999985));
#134483=DIRECTION('center_axis',(0.0522647566817756,0.49726594318179,0.866022503726387));
#134484=DIRECTION('ref_axis',(1.39619082696246E-16,-0.867207748104452,0.497946504785008));
#134485=DIRECTION('center_axis',(-0.055392240656774,-0.527021723598077,
-0.848044693710617));
#134486=DIRECTION('ref_axis',(-0.093152318817715,-0.842916495801014,0.529919264233168));
#134487=DIRECTION('center_axis',(-0.0553922121161263,-0.527021693998996,
-0.848044713969323));
#134488=DIRECTION('ref_axis',(5.85779016094295E-16,0.849348742192404,-0.527832088960287));
#134489=DIRECTION('center_axis',(0.104528463267629,0.994521895368276,6.23081959585229E-15));
#134490=DIRECTION('ref_axis',(0.994521895368276,-0.104528463267629,-4.55502821820944E-30));
#134491=DIRECTION('center_axis',(-0.104528463267628,-0.994521895368276,
-6.94470927749848E-15));
#134492=DIRECTION('ref_axis',(-0.994521895368276,0.104528463267628,-1.09814391166396E-31));
#134493=DIRECTION('center_axis',(0.10452846326765,0.994521895368274,6.95942865237777E-15));
#134494=DIRECTION('ref_axis',(0.994521895368274,-0.10452846326765,-8.52179472506115E-30));
#134495=DIRECTION('center_axis',(0.104528463267629,0.994521895368276,6.23081959585229E-15));
#134496=DIRECTION('ref_axis',(0.994521895368276,-0.104528463267629,-4.55502821820944E-30));
#134497=DIRECTION('center_axis',(0.10452846326765,0.994521895368274,6.95942865237777E-15));
#134498=DIRECTION('ref_axis',(0.994521895368274,-0.10452846326765,-8.52179472506115E-30));
#134499=DIRECTION('center_axis',(-0.0904912830029572,-0.861296695145089,
0.499979330205386));
#134500=DIRECTION('ref_axis',(-0.0513033469950975,-0.497340894869751,-0.866036951219321));
#134501=DIRECTION('center_axis',(0.0522647708473846,0.497266077958568,-0.866022425483298));
#134502=DIRECTION('ref_axis',(9.84167878630125E-17,0.867207670398085,0.497946640115913));
#134503=DIRECTION('center_axis',(0.0522647717855327,0.497266086884299,-0.866022420301566));
#134504=DIRECTION('ref_axis',(-0.994521895368333,0.104528463267083,-3.23450801682927E-13));
#134505=DIRECTION('center_axis',(1.82822378937428E-15,-0.500005014363672,
-0.866022508720867));
#134506=DIRECTION('ref_axis',(1.,-5.03534223352382E-12,2.91979914235583E-12));
#134507=DIRECTION('center_axis',(-3.0042215982928E-5,-0.866018223014645,
-0.500012436349359));
#134508=DIRECTION('ref_axis',(-0.00098970133587607,0.500012217440829,-0.866017784402359));
#134509=DIRECTION('center_axis',(-1.99980824065794E-14,0.500005023014366,
0.86602250372632));
#134510=DIRECTION('ref_axis',(9.19523158479882E-29,-0.86602250372632,0.500005023014366));
#134511=DIRECTION('center_axis',(0.,1.,6.98296267768627E-15));
#134512=DIRECTION('ref_axis',(0.,-6.98296267768627E-15,1.));
#134513=DIRECTION('center_axis',(3.49148133884313E-15,-1.,-6.98296267768627E-15));
#134514=DIRECTION('ref_axis',(-1.,-3.49148133884313E-15,-4.51218105512591E-43));
#134515=DIRECTION('center_axis',(0.,-1.,-6.98296267768627E-15));
#134516=DIRECTION('ref_axis',(0.,6.98296267768627E-15,-1.));
#134517=DIRECTION('center_axis',(3.49148133884313E-15,-1.,-6.98296267768627E-15));
#134518=DIRECTION('ref_axis',(-1.,-3.49148133884313E-15,-4.51218105512591E-43));
#134519=DIRECTION('center_axis',(0.,1.,6.98296267768627E-15));
#134520=DIRECTION('ref_axis',(0.,-6.98296267768627E-15,1.));
#134521=DIRECTION('center_axis',(0.,-0.529924213265795,0.848045003637559));
#134522=DIRECTION('ref_axis',(0.,-0.848045003637559,-0.529924213265795));
#134523=DIRECTION('center_axis',(0.,0.500005158533428,-0.866022425483291));
#134524=DIRECTION('ref_axis',(0.,0.866022425483291,0.500005158533428));
#134525=DIRECTION('center_axis',(-2.16295993207103E-8,0.529924185004342,
-0.848045021297503));
#134526=DIRECTION('ref_axis',(-0.00430950304133444,0.848037146343309,0.529919264233179));
#134527=DIRECTION('center_axis',(0.,-0.529924157141057,0.848045038708641));
#134528=DIRECTION('ref_axis',(0.,-0.848045038708641,-0.529924157141057));
#134529=DIRECTION('center_axis',(-1.05163242810076E-8,0.500005172385359,
-0.866022417485764));
#134530=DIRECTION('ref_axis',(-0.00454855868657297,0.866013458679407,0.500000000000005));
#134531=DIRECTION('center_axis',(3.44576745319419E-5,0.866037336481644,
-0.499979330205208));
#134532=DIRECTION('ref_axis',(0.000963977564194347,0.499979069431728,0.866036951219426));
#134533=DIRECTION('center_axis',(-0.999999970597889,-0.000242495818334613,
-1.35084350642584E-16));
#134534=DIRECTION('ref_axis',(-0.000242495818334613,0.999999970597889,6.82961998416057E-15));
#134535=DIRECTION('center_axis',(3.49148133884313E-15,-1.,-6.98296267768627E-15));
#134536=DIRECTION('ref_axis',(-1.,-3.49148133884313E-15,-4.51218105512591E-43));
#134537=DIRECTION('center_axis',(0.,1.,6.98296267768627E-15));
#134538=DIRECTION('ref_axis',(0.,-6.98296267768627E-15,1.));
#134539=DIRECTION('center_axis',(-1.40816906889911E-16,-6.84214577079636E-15,
1.));
#134540=DIRECTION('ref_axis',(-1.,1.20258066624967E-30,-1.41040152093879E-16));
#134541=DIRECTION('center_axis',(-0.999999970597889,0.000242495818327663,
-1.45036773284147E-16));
#134542=DIRECTION('ref_axis',(0.000242495818327663,0.999999970597889,6.82961998416057E-15));
#134543=DIRECTION('center_axis',(2.89534733035821E-14,0.52992467682556,
0.848044713969332));
#134544=DIRECTION('ref_axis',(-8.01740051201329E-29,-0.848044713969332,
0.52992467682556));
#134545=DIRECTION('center_axis',(-4.63346027506605E-14,0.529924157141126,
-0.848045038708598));
#134546=DIRECTION('ref_axis',(-4.22399707661028E-28,0.848045038708598,0.529924157141126));
#134547=DIRECTION('center_axis',(2.52111351274489E-8,0.529924709439963,
0.8480446935893));
#134548=DIRECTION('ref_axis',(0.00453325469978111,-0.848035979777039,0.529919264233169));
#134549=DIRECTION('center_axis',(4.63345827774717E-14,0.529924742154426,
0.848044673146742));
#134550=DIRECTION('ref_axis',(-4.19038424263683E-28,-0.848044673146742,
0.529924742154426));
#134551=DIRECTION('center_axis',(2.16910432124849E-8,-0.529924185162658,
0.848045021198575));
#134552=DIRECTION('ref_axis',(0.0043095030298541,0.848037146343357,0.529919264233196));
#134553=DIRECTION('center_axis',(0.,0.529924213265795,-0.848045003637559));
#134554=DIRECTION('ref_axis',(0.,0.848045003637559,0.529924213265795));
#134555=DIRECTION('center_axis',(-0.99999996667151,-0.000258180127967688,
-1.61872075241625E-16));
#134556=DIRECTION('ref_axis',(-0.000258180127967688,0.99999996667151,6.82961998416055E-15));
#134557=DIRECTION('center_axis',(0.,1.,6.98296267768627E-15));
#134558=DIRECTION('ref_axis',(0.,-6.98296267768627E-15,1.));
#134559=DIRECTION('center_axis',(-1.40816906889911E-16,-6.84214577079636E-15,
1.));
#134560=DIRECTION('ref_axis',(-1.,8.53463339982835E-31,-1.42635715661134E-16));
#134561=DIRECTION('center_axis',(-0.99999996667151,0.000258180127960702,
-1.44160173554759E-16));
#134562=DIRECTION('ref_axis',(0.000258180127960701,0.99999996667151,6.82961998416055E-15));
#134563=DIRECTION('center_axis',(-3.49148133884313E-15,1.,6.98296267768627E-15));
#134564=DIRECTION('ref_axis',(1.,3.49148133884313E-15,1.12103877145985E-43));
#134565=DIRECTION('center_axis',(-3.00422149895149E-5,0.866018223015033,
0.500012436348687));
#134566=DIRECTION('ref_axis',(-0.000989701305755301,-0.50001221744017,0.866017784402774));
#134567=DIRECTION('center_axis',(0.,-0.529924742154426,-0.848044673146742));
#134568=DIRECTION('ref_axis',(0.,0.848044673146742,-0.529924742154426));
#134569=DIRECTION('center_axis',(-1.01157682251589E-8,-0.500005009599441,
-0.866022511471534));
#134570=DIRECTION('ref_axis',(-0.00447641077753576,-0.86601383461614,0.5));
#134571=DIRECTION('center_axis',(0.,0.500005023014325,0.866022503726343));
#134572=DIRECTION('ref_axis',(0.,-0.866022503726343,0.500005023014325));
#134573=DIRECTION('center_axis',(-2.52907361300284E-8,-0.52992470924582,
-0.848044693710616));
#134574=DIRECTION('ref_axis',(-0.0045332546860101,-0.848035979777084,0.529919264233216));
#134575=DIRECTION('center_axis',(0.,-0.52992467682556,-0.848044713969332));
#134576=DIRECTION('ref_axis',(0.,0.848044713969332,-0.52992467682556));
#134577=DIRECTION('center_axis',(0.,1.,6.98296267768627E-15));
#134578=DIRECTION('ref_axis',(0.,-6.98296267768627E-15,1.));
#134579=DIRECTION('center_axis',(0.,-1.,-6.98296267768627E-15));
#134580=DIRECTION('ref_axis',(0.,6.98296267768627E-15,-1.));
#134581=DIRECTION('center_axis',(-3.49148133884313E-15,1.,6.98296267768627E-15));
#134582=DIRECTION('ref_axis',(1.,3.49148133884313E-15,-5.88545355016423E-44));
#134583=DIRECTION('center_axis',(0.,1.,6.98296267768627E-15));
#134584=DIRECTION('ref_axis',(0.,-6.98296267768627E-15,1.));
#134585=DIRECTION('center_axis',(-3.49148133884313E-15,1.,6.98296267768627E-15));
#134586=DIRECTION('ref_axis',(1.,3.49148133884313E-15,-5.88545355016423E-44));
#134587=DIRECTION('center_axis',(3.44576747051342E-5,-0.866037336481666,
0.499979330205169));
#134588=DIRECTION('ref_axis',(0.000963977560427604,-0.49997906943169,-0.866036951219452));
#134589=DIRECTION('center_axis',(0.,0.500005158533428,-0.866022425483291));
#134590=DIRECTION('ref_axis',(0.,0.866022425483291,0.500005158533428));
#134591=DIRECTION('center_axis',(-1.4393932896948E-15,0.500005167509625,
-0.866022420300809));
#134592=DIRECTION('ref_axis',(-1.,0.,-1.7483827117929E-14));
#134593=DIRECTION('center_axis',(0.0522647557776122,-0.497265934579085,
-0.866022508720585));
#134594=DIRECTION('ref_axis',(0.99452189536815,0.104528463268829,-6.68756390392693E-13));
#134595=DIRECTION('center_axis',(0.0904936763724324,-0.861277224842764,
-0.500012436349085));
#134596=DIRECTION('ref_axis',(-0.053249788326405,0.497169646239297,-0.866017784402541));
#134597=DIRECTION('center_axis',(-0.0522647566818161,0.497265943181915,
0.866022503726313));
#134598=DIRECTION('ref_axis',(-6.22122455512283E-16,-0.867207748104379,
0.497946504785135));
#134599=DIRECTION('center_axis',(-0.104528463267684,0.99452189536827,6.94470927749844E-15));
#134600=DIRECTION('ref_axis',(0.99452189536827,0.104528463267684,4.95746224200719E-30));
#134601=DIRECTION('center_axis',(0.104528463267657,-0.994521895368273,-6.92998990261915E-15));
#134602=DIRECTION('ref_axis',(-0.994521895368273,-0.104528463267657,3.48082151219685E-32));
#134603=DIRECTION('center_axis',(0.104528463267683,-0.99452189536827,-6.94470927749844E-15));
#134604=DIRECTION('ref_axis',(-0.99452189536827,-0.104528463267683,5.29715191372443E-32));
#134605=DIRECTION('center_axis',(0.104528463267657,-0.994521895368273,-6.92998990261915E-15));
#134606=DIRECTION('ref_axis',(-0.994521895368273,-0.104528463267657,3.48082151219685E-32));
#134607=DIRECTION('center_axis',(-0.104528463267683,0.99452189536827,6.94470927749844E-15));
#134608=DIRECTION('ref_axis',(0.99452189536827,0.104528463267683,-5.29715191372443E-32));
#134609=DIRECTION('center_axis',(0.0553921636610116,-0.527021232978663,
0.848045003637544));
#134610=DIRECTION('ref_axis',(5.49983303975455E-17,-0.849349030019346,-0.527831625809971));
#134611=DIRECTION('center_axis',(-0.0522647708473925,0.497266077958566,
-0.866022425483298));
#134612=DIRECTION('ref_axis',(-1.7055667978759E-16,0.867207670398085,0.497946640115912));
#134613=DIRECTION('center_axis',(-0.0553921822241136,0.527021202610446,
-0.848045021297507));
#134614=DIRECTION('ref_axis',(-0.0929299148436241,0.842941044392624,0.529919264233175));
#134615=DIRECTION('center_axis',(0.0553921577943745,-0.52702117716134,0.848045038708652));
#134616=DIRECTION('ref_axis',(3.95891136703E-16,-0.849349064867523,-0.527831569734763));
#134617=DIRECTION('center_axis',(-0.0522647827552366,0.497266090635247,
-0.866022417485764));
#134618=DIRECTION('ref_axis',(-0.0950466972106211,0.860793892490734,0.500000000000003));
#134619=DIRECTION('center_axis',(-0.090491283003073,0.861296695145105,-0.499979330205338));
#134620=DIRECTION('ref_axis',(-0.0513033469963453,0.497340894869573,0.866036951219349));
#134621=DIRECTION('center_axis',(-0.994496518411991,-0.10476962759516,-7.3160239925209E-16));
#134622=DIRECTION('ref_axis',(-0.10476962759516,0.994496518411991,6.82961998416045E-15));
#134623=DIRECTION('center_axis',(0.104528463267657,-0.994521895368273,-6.92998990261915E-15));
#134624=DIRECTION('ref_axis',(-0.994521895368273,-0.104528463267657,3.48082151219685E-32));
#134625=DIRECTION('center_axis',(-0.104528463267683,0.99452189536827,6.94470927749844E-15));
#134626=DIRECTION('ref_axis',(0.99452189536827,0.104528463267683,-5.29715191372443E-32));
#134627=DIRECTION('center_axis',(-1.55536281769218E-16,-6.84291718054622E-15,
1.));
#134628=DIRECTION('ref_axis',(-1.,1.20258066624967E-30,-1.55144167303267E-16));
#134629=DIRECTION('center_axis',(-0.994547213842468,-0.104287292793436,
-7.28234273333503E-16));
#134630=DIRECTION('ref_axis',(-0.104287292793436,0.994547213842468,6.82961998416053E-15));
#134631=DIRECTION('center_axis',(-0.0553922121162014,0.527021693998987,
0.848044713969324));
#134632=DIRECTION('ref_axis',(6.84979756801523E-16,-0.849348742192409,0.527832088960281));
#134633=DIRECTION('center_axis',(-0.0553921577943754,0.527021177161349,
-0.848045038708646));
#134634=DIRECTION('ref_axis',(-2.883936554783E-16,0.849349064867518,0.527831569734772));
#134635=DIRECTION('center_axis',(-0.0553921904533803,0.527021729069898,
0.848044693589289));
#134636=DIRECTION('ref_axis',(0.0931523188159149,-0.84291649580119,0.529919264233203));
#134637=DIRECTION('center_axis',(-0.0553922189449272,0.527021758969973,
0.848044673146735));
#134638=DIRECTION('ref_axis',(1.27494230359798E-16,-0.849348701629309,0.527832154231444));
#134639=DIRECTION('center_axis',(0.0553921822969478,-0.527021202762016,
0.848045021198556));
#134640=DIRECTION('ref_axis',(-0.0843581245706196,0.843841975854163,0.529919264233213));
#134641=DIRECTION('center_axis',(-0.0553921636610064,0.527021232978614,
-0.848045003637574));
#134642=DIRECTION('ref_axis',(5.9573696388713E-16,0.849349030019376,0.527831625809922));
#134643=DIRECTION('center_axis',(-0.994494875050338,-0.10478522557409,-7.31711319356807E-16));
#134644=DIRECTION('ref_axis',(-0.10478522557409,0.994494875050338,6.82961998416065E-15));
#134645=DIRECTION('center_axis',(-0.104528463267683,0.99452189536827,6.94470927749844E-15));
#134646=DIRECTION('ref_axis',(0.99452189536827,0.104528463267683,2.7081584375864E-32));
#134647=DIRECTION('center_axis',(-1.55536281769218E-16,-6.84291718054622E-15,
1.));
#134648=DIRECTION('ref_axis',(-1.,1.28019500997425E-30,-1.576500015202E-16));
#134649=DIRECTION('center_axis',(-0.994548849394382,-0.104271693993676,
-7.28125347496963E-16));
#134650=DIRECTION('ref_axis',(-0.104271693993676,0.994548849394382,6.8296199841608E-15));
#134651=DIRECTION('center_axis',(-0.104528463267657,0.994521895368273,6.92998990261915E-15));
#134652=DIRECTION('ref_axis',(0.994521895368273,0.104528463267657,8.40007115892777E-30));
#134653=DIRECTION('center_axis',(-0.0905534316544792,0.861270944309615,
0.500012436348959));
#134654=DIRECTION('ref_axis',(0.0512812290718702,-0.497376550154188,0.866017784402605));
#134655=DIRECTION('center_axis',(0.0553922189449268,-0.527021758969966,
-0.84804467314674));
#134656=DIRECTION('ref_axis',(-2.83402997067715E-16,0.849348701629314,-0.527832154231436));
#134657=DIRECTION('center_axis',(0.0522647452180362,-0.497265930897975,
-0.866022511471535));
#134658=DIRECTION('ref_axis',(0.0860712067675025,-0.861737632557378,0.499999999999992));
#134659=DIRECTION('center_axis',(-0.0522647566818046,0.497265943181806,
0.866022503726376));
#134660=DIRECTION('ref_axis',(-3.85785311454816E-16,-0.867207748104442,
0.497946504785025));
#134661=DIRECTION('center_axis',(0.0553921903485681,-0.527021728885636,
-0.848044693710646));
#134662=DIRECTION('ref_axis',(0.0841354767001877,-0.843864204096268,0.529919264233152));
#134663=DIRECTION('center_axis',(0.0553922121161999,-0.527021693998973,
-0.848044713969333));
#134664=DIRECTION('ref_axis',(6.18235216948487E-16,0.849348742192417,-0.527832088960266));
#134665=DIRECTION('center_axis',(-0.104528463267683,0.99452189536827,6.94470927749844E-15));
#134666=DIRECTION('ref_axis',(0.99452189536827,0.104528463267683,2.7081584375864E-32));
#134667=DIRECTION('center_axis',(0.104528463267682,-0.99452189536827,-6.94470927749844E-15));
#134668=DIRECTION('ref_axis',(-0.99452189536827,-0.104528463267682,4.98335217676857E-30));
#134669=DIRECTION('center_axis',(-0.104528463267657,0.994521895368273,6.92998990261915E-15));
#134670=DIRECTION('ref_axis',(0.994521895368273,0.104528463267657,8.40007115892777E-30));
#134671=DIRECTION('center_axis',(-0.104528463267683,0.99452189536827,6.19962518494839E-14));
#134672=DIRECTION('ref_axis',(0.99452189536827,0.104528463267683,3.69415865639377E-31));
#134673=DIRECTION('center_axis',(-0.104528463267657,0.994521895368273,6.92998990261915E-15));
#134674=DIRECTION('ref_axis',(0.994521895368273,0.104528463267657,8.40007115892777E-30));
#134675=DIRECTION('center_axis',(0.0905598208266182,-0.861289491529548,
0.499979330205383));
#134676=DIRECTION('ref_axis',(0.0532207405915228,-0.497139368682093,-0.866036951219323));
#134677=DIRECTION('center_axis',(-0.0522647708474152,0.4972660779586,-0.866022425483278));
#134678=DIRECTION('ref_axis',(3.08393337172386E-16,0.867207670398066,0.497946640115946));
#134679=DIRECTION('center_axis',(-0.0522647717851799,0.497266086880897,
-0.866022420303541));
#134680=DIRECTION('ref_axis',(-0.994521895368013,-0.104528463270131,-1.43804478045958E-12));
#134681=DIRECTION('center_axis',(0.103956887953212,-0.4890787051524,-0.866022508722225));
#134682=DIRECTION('ref_axis',(0.978147600733671,0.207911690818393,-3.89015155196725E-13));
#134683=DIRECTION('center_axis',(0.180025927304702,-0.847099893161453,-0.500012436349274));
#134684=DIRECTION('ref_axis',(-0.104926459543619,0.488879980349352,-0.86601778440241));
#134685=DIRECTION('center_axis',(-0.103956889752312,0.489078713616365,0.866022503726311));
#134686=DIRECTION('ref_axis',(1.64971394491684E-16,-0.870740345484705,0.491743073916834));
#134687=DIRECTION('center_axis',(-0.207911690817751,0.978147600733807,6.83036818919254E-15));
#134688=DIRECTION('ref_axis',(0.978147600733807,0.207911690817751,-3.90426835043966E-29));
#134689=DIRECTION('center_axis',(0.207911690817763,-0.978147600733805,-6.80109070798532E-15));
#134690=DIRECTION('ref_axis',(-0.978147600733805,-0.207911690817763,2.97563208683757E-32));
#134691=DIRECTION('center_axis',(0.207911690817757,-0.978147600733806,-3.99045251209326E-15));
#134692=DIRECTION('ref_axis',(-0.978147600733806,-0.207911690817757,7.01829476299402E-32));
#134693=DIRECTION('center_axis',(0.207911690817763,-0.978147600733805,-6.80109070798532E-15));
#134694=DIRECTION('ref_axis',(-0.978147600733805,-0.207911690817763,2.97563208683757E-32));
#134695=DIRECTION('center_axis',(-0.207911690817757,0.978147600733806,6.83036818919254E-15));
#134696=DIRECTION('ref_axis',(0.978147600733806,0.207911690817757,-2.9624920046404E-32));
#134697=DIRECTION('center_axis',(0.110177439185365,-0.518344097776712,0.848045003637544));
#134698=DIRECTION('ref_axis',(-2.27092564730572E-16,-0.853239582811832,
-0.521519140898099));
#134699=DIRECTION('center_axis',(-0.103956917928266,0.489078846174011,-0.866022425483286));
#134700=DIRECTION('ref_axis',(3.62085698470434E-16,0.870740269393772,0.491743208652709));
#134701=DIRECTION('center_axis',(-0.110177454465313,0.518344065636003,-0.848045021297503));
#134702=DIRECTION('ref_axis',(-0.180532167021475,0.82860950396738,0.529919264233207));
#134703=DIRECTION('center_axis',(0.110177427516371,-0.518344042878409,0.848045038708641));
#134704=DIRECTION('ref_axis',(-7.51351770475333E-16,-0.853239616987296,
-0.521519084984789));
#134705=DIRECTION('center_axis',(-0.103956931087326,0.489078857538383,-0.866022417485746));
#134706=DIRECTION('ref_axis',(-0.184503484218911,0.846143288285776,0.500000000000017));
#134707=DIRECTION('center_axis',(-0.180025582247482,0.847119506978703,-0.499979330205374));
#134708=DIRECTION('ref_axis',(-0.103008581351147,0.489253749388556,0.866036951219325));
#134709=DIRECTION('center_axis',(-0.978097154258593,-0.208148881407615,
-1.45349587027152E-15));
#134710=DIRECTION('ref_axis',(-0.208148881407615,0.978097154258593,6.82961998416083E-15));
#134711=DIRECTION('center_axis',(0.207911690817763,-0.978147600733805,-6.80109070798532E-15));
#134712=DIRECTION('ref_axis',(-0.978147600733805,-0.207911690817763,2.97563208683757E-32));
#134713=DIRECTION('center_axis',(-0.207911690817757,0.978147600733806,6.83036818919254E-15));
#134714=DIRECTION('ref_axis',(0.978147600733806,0.207911690817757,-2.9624920046404E-32));
#134715=DIRECTION('center_axis',(-1.70094388097119E-16,-6.84522295806915E-15,
1.));
#134716=DIRECTION('ref_axis',(-1.,1.20258066624967E-30,-1.69248182512655E-16));
#134717=DIRECTION('center_axis',(-0.978197989689808,-0.20767448800182,-1.45018319882431E-15));
#134718=DIRECTION('ref_axis',(-0.20767448800182,0.978197989689808,6.82961998416085E-15));
#134719=DIRECTION('center_axis',(-0.110177535564866,0.518344551206608,0.848044713969301));
#134720=DIRECTION('ref_axis',(2.46979766523084E-16,-0.853239300541025,0.521519602711406));
#134721=DIRECTION('center_axis',(-0.110177427516374,0.518344042878427,-0.84804503870863));
#134722=DIRECTION('ref_axis',(1.47794069500662E-15,0.853239616987286,0.521519084984807));
#134723=DIRECTION('center_axis',(-0.110177517688164,0.518344588349403,0.848044693589296));
#134724=DIRECTION('ref_axis',(0.180750786632584,-0.828561842306435,0.529919264233211));
#134725=DIRECTION('center_axis',(-0.110177549147463,0.518344615107834,0.848044673146745));
#134726=DIRECTION('ref_axis',(-1.32855656284121E-15,-0.853239260760977,
0.521519667794093));
#134727=DIRECTION('center_axis',(0.110177454563686,-0.518344065776971,0.84804502119856));
#134728=DIRECTION('ref_axis',(-0.172101506913406,0.830401496092503,0.529919264233211));
#134729=DIRECTION('center_axis',(-0.110177439185362,0.518344097776696,-0.848045003637554));
#134730=DIRECTION('ref_axis',(-1.92246784709572E-16,0.853239582811842,0.521519140898083));
#134731=DIRECTION('center_axis',(-0.978093889466682,-0.208164222161104,
-1.45360299418058E-15));
#134732=DIRECTION('ref_axis',(-0.208164222161104,0.978093889466682,6.82961998416055E-15));
#134733=DIRECTION('center_axis',(-0.207911690817757,0.978147600733806,6.83036818919254E-15));
#134734=DIRECTION('ref_axis',(0.978147600733806,0.207911690817757,-2.70700739195018E-31));
#134735=DIRECTION('center_axis',(-1.70094388097119E-16,-6.84522295806915E-15,
1.));
#134736=DIRECTION('ref_axis',(-1.,1.28019500997425E-30,-1.72664287379267E-16));
#134737=DIRECTION('center_axis',(-0.978201246800563,-0.207659145615656,
-1.45007606351434E-15));
#134738=DIRECTION('ref_axis',(-0.207659145615656,0.978201246800563,6.82961998416061E-15));
#134739=DIRECTION('center_axis',(-0.207911690817763,0.978147600733805,6.80109070798532E-15));
#134740=DIRECTION('ref_axis',(0.978147600733805,0.207911690817763,-4.42525447058535E-29));
#134741=DIRECTION('center_axis',(-0.18008469874793,0.847087400905451,0.500012436349452));
#134742=DIRECTION('ref_axis',(0.10299031155993,-0.489291521307827,0.866017784402296));
#134743=DIRECTION('center_axis',(0.110177549147566,-0.518344615107816,-0.848044673146743));
#134744=DIRECTION('ref_axis',(8.16820715362172E-16,0.853239260760984,-0.521519667794082));
#134745=DIRECTION('center_axis',(0.103956877076738,-0.489078702596054,-0.866022511471505));
#134746=DIRECTION('ref_axis',(0.175675810171962,-0.848020052664076,0.500000000000043));
#134747=DIRECTION('center_axis',(-0.103956889752265,0.489078713616238,0.866022503726388));
#134748=DIRECTION('ref_axis',(1.0747599324937E-15,-0.870740345484778,0.491743073916704));
#134749=DIRECTION('center_axis',(0.1101775175661,-0.518344588176855,-0.848044693710619));
#134750=DIRECTION('ref_axis',(0.1718824022104,-0.83044687560673,0.52991926423315));
#134751=DIRECTION('center_axis',(0.110177535564884,-0.518344551206552,-0.848044713969332));
#134752=DIRECTION('ref_axis',(9.13576263120513E-16,0.853239300541059,-0.521519602711351));
#134753=DIRECTION('center_axis',(-0.207911690817757,0.978147600733806,9.67028386629181E-15));
#134754=DIRECTION('ref_axis',(0.978147600733806,0.207911690817757,-3.68301291740874E-31));
#134755=DIRECTION('center_axis',(0.207911690817754,-0.978147600733807,-6.83036818919254E-15));
#134756=DIRECTION('ref_axis',(-0.978147600733807,-0.207911690817754,1.95800148050649E-29));
#134757=DIRECTION('center_axis',(-0.207911690817763,0.978147600733805,6.80109070798532E-15));
#134758=DIRECTION('ref_axis',(0.978147600733805,0.207911690817763,-4.42525447058535E-29));
#134759=DIRECTION('center_axis',(-0.207911690817757,0.978147600733806,2.67097779288864E-14));
#134760=DIRECTION('ref_axis',(0.978147600733806,0.207911690817757,2.13282960949029E-31));
#134761=DIRECTION('center_axis',(-0.207911690817763,0.978147600733805,6.80109070798532E-15));
#134762=DIRECTION('ref_axis',(0.978147600733805,0.207911690817763,-4.42525447058535E-29));
#134763=DIRECTION('center_axis',(0.180092991631071,-0.847105178672037,0.499979330205147));
#134764=DIRECTION('ref_axis',(0.104894406048821,-0.488852904974673,-0.866036951219455));
#134765=DIRECTION('center_axis',(-0.10395691792829,0.489078846174027,-0.866022425483274));
#134766=DIRECTION('ref_axis',(6.38663846784148E-16,0.870740269393762,0.491743208652727));
#134767=DIRECTION('center_axis',(-0.103956919793601,0.489078854949547,-0.866022420303462));
#134768=DIRECTION('ref_axis',(-0.978147600732871,-0.207911690822154,-2.56575162955948E-12));
#134769=DIRECTION('center_axis',(0.154510046709071,-0.475533027084736,-0.866022508724565));
#134770=DIRECTION('ref_axis',(0.951056516293718,0.309016994379366,-2.70999321601511E-12));
#134771=DIRECTION('center_axis',(0.267585776505254,-0.823641557784567,-0.50001243634763));
#134772=DIRECTION('ref_axis',(-0.155453534437441,0.475234043107105,-0.866017784403404));
#134773=DIRECTION('center_axis',(-0.154510049384291,0.475533035318136,0.866022503726309));
#134774=DIRECTION('ref_axis',(-1.56718497740608E-15,-0.876548788012437,
0.481313018974064));
#134775=DIRECTION('center_axis',(-0.309016994374972,0.951056516295146,6.64119215765932E-15));
#134776=DIRECTION('ref_axis',(0.951056516295146,0.309016994374972,3.41480999208037E-15));
#134777=DIRECTION('center_axis',(0.309016994374951,-0.951056516295152,-6.59767734033507E-15));
#134778=DIRECTION('ref_axis',(-0.951056516295152,-0.309016994374951,-3.41480999208033E-15));
#134779=DIRECTION('center_axis',(0.309016994374964,-0.951056516295148,-6.64119215765934E-15));
#134780=DIRECTION('ref_axis',(-0.951056516295148,-0.309016994374964,-3.41480999208031E-15));
#134781=DIRECTION('center_axis',(0.309016994374951,-0.951056516295152,-6.59767734033507E-15));
#134782=DIRECTION('ref_axis',(-0.951056516295152,-0.309016994374951,-3.41480999208033E-15));
#134783=DIRECTION('center_axis',(-0.309016994374922,0.951056516295162,6.64119215765944E-15));
#134784=DIRECTION('ref_axis',(0.951056516295162,0.309016994374922,3.41480999208039E-15));
#134785=DIRECTION('center_axis',(0.163755587629901,-0.503987876168983,0.84804500363758));
#134786=DIRECTION('ref_axis',(2.36007916206428E-16,-0.859649462041489,-0.510884333691863));
#134787=DIRECTION('center_axis',(-0.154510091261978,0.475533164204401,-0.866022425483293));
#134788=DIRECTION('ref_axis',(2.20635803329686E-16,0.876548714628842,0.481313152617426));
#134789=DIRECTION('center_axis',(-0.163755599470739,0.503987842605832,-0.848045021297512));
#134790=DIRECTION('ref_axis',(-0.266156471022805,0.805199544415683,0.529919264233206));
#134791=DIRECTION('center_axis',(0.163755570286413,-0.503987822791216,0.848045038708642));
#134792=DIRECTION('ref_axis',(1.41142713906073E-15,-0.859649495083696,-0.510884278092747));
#134793=DIRECTION('center_axis',(-0.154510105538923,0.475533174130323,-0.866022417485766));
#134794=DIRECTION('ref_axis',(-0.271938812460818,0.822222161144676,0.499999999999979));
#134795=DIRECTION('center_axis',(-0.267587483539841,0.823661100222957,-0.499979330205082));
#134796=DIRECTION('ref_axis',(-0.153585232147035,0.475806237442058,0.866036951219504));
#134797=DIRECTION('center_axis',(-0.950981553003154,-0.309247612517397,
-2.15946453637257E-15));
#134798=DIRECTION('ref_axis',(-0.309247612517397,0.950981553003154,6.82961998416078E-15));
#134799=DIRECTION('center_axis',(0.309016994374951,-0.951056516295152,-6.59767734033507E-15));
#134800=DIRECTION('ref_axis',(-0.951056516295152,-0.309016994374951,-3.41480999208033E-15));
#134801=DIRECTION('center_axis',(-0.309016994374972,0.951056516295146,6.64119215765932E-15));
#134802=DIRECTION('ref_axis',(0.951056516295146,0.309016994374972,3.41480999208037E-15));
#134803=DIRECTION('center_axis',(-1.84331724214208E-16,-6.84903784078409E-15,
1.));
#134804=DIRECTION('ref_axis',(-1.,1.20258066624967E-30,-1.83352197722043E-16));
#134805=DIRECTION('center_axis',(-0.951131423661017,-0.308786358060986,
-2.15624361371854E-15));
#134806=DIRECTION('ref_axis',(-0.308786358060986,0.951131423661017,6.82961998416067E-15));
#134807=DIRECTION('center_axis',(-0.163755730877694,0.50398831704057,0.848044713969332));
#134808=DIRECTION('ref_axis',(4.71763757776837E-17,-0.859649189130476,0.510884792910609));
#134809=DIRECTION('center_axis',(-0.163755570286353,0.503987822791179,-0.848045038708675));
#134810=DIRECTION('ref_axis',(1.32327065984906E-15,0.859649495083721,0.510884278092704));
#134811=DIRECTION('center_axis',(-0.163755716975923,0.503988355850381,0.848044693589277));
#134812=DIRECTION('ref_axis',(0.266368911021071,-0.805129291875531,0.5299192642332));
#134813=DIRECTION('center_axis',(-0.163755751065448,0.503988379172,0.848044673146746));
#134814=DIRECTION('ref_axis',(-2.31894814760129E-15,-0.859649150669469,
0.510884857627685));
#134815=DIRECTION('center_axis',(0.163755599576039,-0.503987842738117,0.848045021198563));
#134816=DIRECTION('ref_axis',(-0.25795930914358,0.80786296376346,0.529919264233228));
#134817=DIRECTION('center_axis',(-0.163755587629911,0.503987876169013,-0.848045003637561));
#134818=DIRECTION('ref_axis',(1.28133843970483E-15,0.859649462041471,0.510884333691894));
#134819=DIRECTION('center_axis',(-0.950976702550718,-0.309262527968978,
-1.12416423283092E-14));
#134820=DIRECTION('ref_axis',(-0.309262527968978,0.950976702550718,6.82961998416086E-15));
#134821=DIRECTION('center_axis',(-0.309016994374964,0.951056516295148,6.64119215765934E-15));
#134822=DIRECTION('ref_axis',(0.951056516295148,0.309016994374964,3.41480999208031E-15));
#134823=DIRECTION('center_axis',(-1.84331724214208E-16,-6.84903784078409E-15,
1.));
#134824=DIRECTION('ref_axis',(-1.,1.28019500997425E-30,-1.87678573238334E-16));
#134825=DIRECTION('center_axis',(-0.951136266645025,-0.308771440182806,
-2.15613944273197E-15));
#134826=DIRECTION('ref_axis',(-0.308771440182806,0.951136266645025,6.82961998416067E-15));
#134827=DIRECTION('center_axis',(-0.309016994374951,0.951056516295152,6.59767734033507E-15));
#134828=DIRECTION('ref_axis',(0.951056516295152,0.309016994374951,3.41480999208041E-15));
#134829=DIRECTION('center_axis',(-0.267642920196027,0.823622990672906,0.500012436349299));
#134830=DIRECTION('ref_axis',(0.153571010712917,-0.475845712145576,0.866017784402424));
#134831=DIRECTION('center_axis',(0.163755751065493,-0.503988379172002,-0.848044673146736));
#134832=DIRECTION('ref_axis',(-1.92007597614245E-15,0.859649150669465,-0.510884857627692));
#134833=DIRECTION('center_axis',(0.154510035625077,-0.475533025683493,-0.866022511471521));
#134834=DIRECTION('ref_axis',(0.26335567262561,-0.825011387615885,0.500000000000024));
#134835=DIRECTION('center_axis',(-0.154510049384261,0.475533035318041,0.866022503726367));
#134836=DIRECTION('ref_axis',(-1.66937126522959E-15,-0.876548788012491,
0.481313018973965));
#134837=DIRECTION('center_axis',(0.163755716841192,-0.503988355689969,-0.848044693710625));
#134838=DIRECTION('ref_axis',(0.257746148176438,-0.807930997359779,0.529919264233187));
#134839=DIRECTION('center_axis',(0.163755730877767,-0.503988317040554,-0.848044713969328));
#134840=DIRECTION('ref_axis',(-4.27283864732672E-16,0.859649189130481,-0.510884792910599));
#134841=DIRECTION('center_axis',(-0.309016994374964,0.951056516295148,6.64119215765934E-15));
#134842=DIRECTION('ref_axis',(0.951056516295148,0.309016994374964,3.41480999208031E-15));
#134843=DIRECTION('center_axis',(0.309016994374964,-0.951056516295148,-6.64119215765934E-15));
#134844=DIRECTION('ref_axis',(-0.951056516295148,-0.309016994374964,-3.41480999208031E-15));
#134845=DIRECTION('center_axis',(-0.309016994374951,0.951056516295152,6.59767734033507E-15));
#134846=DIRECTION('ref_axis',(0.951056516295152,0.309016994374951,3.41480999208041E-15));
#134847=DIRECTION('center_axis',(-0.309016994374964,0.951056516295148,7.54877779975346E-14));
#134848=DIRECTION('ref_axis',(0.951056516295148,0.309016994374964,3.41480999207973E-15));
#134849=DIRECTION('center_axis',(-0.309016994374951,0.951056516295152,6.59767734033507E-15));
#134850=DIRECTION('ref_axis',(0.951056516295152,0.309016994374951,3.41480999208041E-15));
#134851=DIRECTION('center_axis',(0.267653025932096,-0.823639804208751,0.499979330205123));
#134852=DIRECTION('ref_axis',(0.15541882643867,-0.475210466541842,-0.866036951219468));
#134853=DIRECTION('center_axis',(-0.154510091261975,0.475533164204405,-0.866022425483291));
#134854=DIRECTION('ref_axis',(4.76968987462892E-16,0.87654871462884,0.48131315261743));
#134855=DIRECTION('center_axis',(-0.154510094034918,0.47553317273861,-0.866022420302426));
#134856=DIRECTION('ref_axis',(-0.951056516295898,-0.309016994372655,1.39870616942708E-12));
#134857=DIRECTION('center_axis',(0.203370361064571,-0.456777309673213,-0.866022508719126));
#134858=DIRECTION('ref_axis',(0.913545457644057,0.406736643072529,2.07183352317727E-12));
#134859=DIRECTION('center_axis',(0.352213899943352,-0.791159233140772,-0.500012436348137));
#134860=DIRECTION('ref_axis',(-0.204277427961519,0.456381342216139,-0.866017784403081));
#134861=DIRECTION('center_axis',(-0.203370364581912,0.456777317573267,0.866022503726313));
#134862=DIRECTION('ref_axis',(1.2472944269153E-15,-0.884507036382102,0.466526850878437));
#134863=DIRECTION('center_axis',(-0.406736643075807,0.913545457642598,6.37925383508808E-15));
#134864=DIRECTION('ref_axis',(0.913545457642598,0.406736643075807,3.4148099920803E-15));
#134865=DIRECTION('center_axis',(0.406736643075804,-0.913545457642599,-6.32197843909137E-15));
#134866=DIRECTION('ref_axis',(-0.913545457642599,-0.406736643075804,-3.41480999208033E-15));
#134867=DIRECTION('center_axis',(0.406736643075807,-0.913545457642598,-6.37925383508808E-15));
#134868=DIRECTION('ref_axis',(-0.913545457642598,-0.406736643075807,-3.4148099920803E-15));
#134869=DIRECTION('center_axis',(0.406736643075804,-0.913545457642599,-6.32197843909137E-15));
#134870=DIRECTION('ref_axis',(-0.913545457642599,-0.406736643075804,-3.41480999208033E-15));
#134871=DIRECTION('center_axis',(-0.406736643075817,0.913545457642594,6.37925383508805E-15));
#134872=DIRECTION('ref_axis',(0.913545457642593,0.406736643075817,3.41480999208037E-15));
#134873=DIRECTION('center_axis',(0.215539595588306,-0.484109857923776,0.848045003637573));
#134874=DIRECTION('ref_axis',(-8.96693424359429E-16,-0.868458021515992,
-0.495762710240019));
#134875=DIRECTION('center_axis',(-0.203370419702479,0.45677744137614,-0.866022425483258));
#134876=DIRECTION('ref_axis',(5.21321035819439E-17,0.884506966812022,0.466526982779128));
#134877=DIRECTION('center_axis',(-0.215539603846564,0.484109823311004,-0.848045021297487));
#134878=DIRECTION('ref_axis',(-0.348864709038018,0.77296765015256,0.529919264233192));
#134879=DIRECTION('center_axis',(0.215539572760321,-0.484109806651282,0.848045038708651));
#134880=DIRECTION('ref_axis',(1.04124665764134E-15,-0.868458052949961,-0.495762655175199));
#134881=DIRECTION('center_axis',(-0.203370434945702,0.456777449752215,-0.866022417485748));
#134882=DIRECTION('ref_axis',(-0.356394722164787,0.789292595944645,0.500000000000047));
#134883=DIRECTION('center_axis',(-0.35221764036688,0.791178490090346,-0.499979330205507));
#134884=DIRECTION('ref_axis',(-0.202479170976877,0.457145692797587,0.866036951219248));
#134885=DIRECTION('center_axis',(-0.913446798847324,-0.406958162070226,
-2.84177365711619E-15));
#134886=DIRECTION('ref_axis',(-0.406958162070226,0.913446798847324,6.82961998416052E-15));
#134887=DIRECTION('center_axis',(0.406736643075804,-0.913545457642599,-6.32197843909137E-15));
#134888=DIRECTION('ref_axis',(-0.913545457642599,-0.406736643075804,-3.41480999208033E-15));
#134889=DIRECTION('center_axis',(-0.406736643075817,0.913545457642594,6.37925383508805E-15));
#134890=DIRECTION('ref_axis',(0.913545457642593,0.406736643075817,3.41480999208037E-15));
#134891=DIRECTION('center_axis',(-1.98092302886631E-16,-6.85432003203771E-15,
1.));
#134892=DIRECTION('ref_axis',(-1.,1.60344088833289E-30,-1.97456212931431E-16));
#134893=DIRECTION('center_axis',(-0.913644062717546,-0.406515100163544,
-2.83867977235792E-15));
#134894=DIRECTION('ref_axis',(-0.406515100163544,0.913644062717546,6.82961998416061E-15));
#134895=DIRECTION('center_axis',(-0.21553978413504,0.484110281406725,0.84804471396933));
#134896=DIRECTION('ref_axis',(1.68002389095411E-15,-0.868457761888284,0.495763165045561));
#134897=DIRECTION('center_axis',(-0.215539572760312,0.48410980665126,-0.848045038708666));
#134898=DIRECTION('ref_axis',(-2.44700238975538E-15,0.868458052949974,0.495762655175175));
#134899=DIRECTION('center_axis',(-0.215539774366204,0.484110321457017,0.848044693589288));
#134900=DIRECTION('ref_axis',(0.349068641889459,-0.772875576431343,0.529919264233116));
#134901=DIRECTION('center_axis',(-0.215539810706662,0.484110341087615,0.848044673146745));
#134902=DIRECTION('ref_axis',(8.10725224855173E-16,-0.86845772529927,0.495763229140704));
#134903=DIRECTION('center_axis',(0.215539603979383,-0.484109823425178,0.848045021198553));
#134904=DIRECTION('ref_axis',(-0.340990855174767,0.776473315756408,0.529919264233177));
#134905=DIRECTION('center_axis',(-0.215539595588304,0.484109857923771,-0.848045003637576));
#134906=DIRECTION('ref_axis',(3.1646774827737E-16,0.868458021515995,0.495762710240014));
#134907=DIRECTION('center_axis',(-0.913440415876946,-0.406972488803054,
-2.50776132404211E-14));
#134908=DIRECTION('ref_axis',(-0.406972488803054,0.913440415876946,6.82961998416034E-15));
#134909=DIRECTION('center_axis',(-0.406736643075807,0.913545457642598,1.74906806584517E-14));
#134910=DIRECTION('ref_axis',(0.913545457642598,0.406736643075807,3.4148099920803E-15));
#134911=DIRECTION('center_axis',(-1.98092302886631E-16,-6.85432003203771E-15,
1.));
#134912=DIRECTION('ref_axis',(-1.,1.28019500997425E-30,-1.95185716167867E-16));
#134913=DIRECTION('center_axis',(-0.913650438514062,-0.40650077023674,-2.83857970701388E-15));
#134914=DIRECTION('ref_axis',(-0.40650077023674,0.913650438514061,6.8296199841608E-15));
#134915=DIRECTION('center_axis',(-0.406736643075804,0.913545457642599,6.32197843909137E-15));
#134916=DIRECTION('ref_axis',(0.913545457642599,0.406736643075804,3.41480999208028E-15));
#134917=DIRECTION('center_axis',(-0.352268789800574,0.791134794601461,0.500012436348681));
#134918=DIRECTION('ref_axis',(0.202469153692002,-0.457186437792438,0.866017784402783));
#134919=DIRECTION('center_axis',(0.215539810706706,-0.4841103410876,-0.848044673146743));
#134920=DIRECTION('ref_axis',(-1.47259052727932E-15,0.868457725299275,-0.495763229140694));
#134921=DIRECTION('center_axis',(0.203370349883188,-0.456777309433043,-0.866022511471555));
#134922=DIRECTION('ref_axis',(0.348150155221207,-0.792963725159901,0.499999999999983));
#134923=DIRECTION('center_axis',(-0.203370364581871,0.456777317573174,0.866022503726371));
#134924=DIRECTION('ref_axis',(1.52619955059002E-15,-0.884507036382154,0.466526850878339));
#134925=DIRECTION('center_axis',(0.215539774217316,-0.484110321310761,-0.848044693710621));
#134926=DIRECTION('ref_axis',(0.340785973383427,-0.776563258041277,0.529919264233172));
#134927=DIRECTION('center_axis',(0.215539784135144,-0.484110281406682,-0.848044713969328));
#134928=DIRECTION('ref_axis',(1.69535706659914E-15,0.868457761888303,-0.495763165045528));
#134929=DIRECTION('center_axis',(-0.406736643075807,0.913545457642598,6.37925383508808E-15));
#134930=DIRECTION('ref_axis',(0.913545457642598,0.406736643075807,3.4148099920803E-15));
#134931=DIRECTION('center_axis',(0.406736643075807,-0.913545457642598,-6.37925383508808E-15));
#134932=DIRECTION('ref_axis',(-0.913545457642598,-0.406736643075807,-3.4148099920803E-15));
#134933=DIRECTION('center_axis',(-0.406736643075804,0.913545457642599,6.32197843909137E-15));
#134934=DIRECTION('ref_axis',(0.913545457642599,0.406736643075804,3.41480999208028E-15));
#134935=DIRECTION('center_axis',(-0.406736643075807,0.913545457642598,-1.58435998116392E-14));
#134936=DIRECTION('ref_axis',(0.913545457642598,0.406736643075807,3.4148099920803E-15));
#134937=DIRECTION('center_axis',(-0.406736643075804,0.913545457642599,6.32197843909137E-15));
#134938=DIRECTION('ref_axis',(0.913545457642599,0.406736643075804,3.41480999208028E-15));
#134939=DIRECTION('center_axis',(0.352280597671406,-0.791150459692788,0.499979330204927));
#134940=DIRECTION('ref_axis',(0.204240445639035,-0.456361522794654,-0.866036951219584));
#134941=DIRECTION('center_axis',(-0.203370419702479,0.4567774413761,-0.866022425483279));
#134942=DIRECTION('ref_axis',(-2.08635189661219E-15,0.884506966812044,0.466526982779087));
#134943=DIRECTION('center_axis',(-0.203370423353607,0.456777449576576,-0.866022420300591));
#134944=DIRECTION('ref_axis',(-0.913545457644566,-0.406736643071388,2.81926712275846E-12));
#134945=DIRECTION('center_axis',(0.250002507180728,-0.433017044456612,-0.866022508722152));
#134946=DIRECTION('ref_axis',(0.866025403787112,0.49999999999537,3.0815245439773E-12));
#134947=DIRECTION('center_axis',(0.432983094187539,-0.750008802379581,-0.500012436346269));
#134948=DIRECTION('ref_axis',(-0.250863215247079,0.432528431818864,-0.866017784404115));
#134949=DIRECTION('center_axis',(-0.250002511507198,0.433017051950273,0.866022503726311));
#134950=DIRECTION('ref_axis',(-4.23904869311635E-16,-0.894424794863787,
0.447218387740121));
#134951=DIRECTION('center_axis',(-0.499999999999998,0.86602540378444,6.70236582766913E-14));
#134952=DIRECTION('ref_axis',(0.86602540378444,0.499999999999998,3.41480999207943E-15));
#134953=DIRECTION('center_axis',(0.500000000000004,-0.866025403784436,-5.97701461910994E-15));
#134954=DIRECTION('ref_axis',(-0.866025403784436,-0.500000000000004,-3.41480999208033E-15));
#134955=DIRECTION('center_axis',(0.50000000000001,-0.866025403784433,-6.04742307255487E-15));
#134956=DIRECTION('ref_axis',(-0.866025403784433,-0.50000000000001,-3.41480999208034E-15));
#134957=DIRECTION('center_axis',(0.500000000000004,-0.866025403784436,-5.97701461910994E-15));
#134958=DIRECTION('ref_axis',(-0.866025403784436,-0.500000000000004,-3.41480999208033E-15));
#134959=DIRECTION('center_axis',(-0.50000000000001,0.866025403784433,6.04742307255487E-15));
#134960=DIRECTION('ref_axis',(0.866025403784433,0.50000000000001,3.41480999208034E-15));
#134961=DIRECTION('center_axis',(0.264962106632886,-0.458927830768649,0.84804500363757));
#134962=DIRECTION('ref_axis',(-1.55726465520226E-15,-0.879478602053318,
-0.475938429348105));
#134963=DIRECTION('center_axis',(-0.250002579266717,0.433017169313229,-0.866022425483282));
#134964=DIRECTION('ref_axis',(-1.52069700702419E-17,0.89442473021641,0.447218517033119));
#134965=DIRECTION('center_axis',(-0.264962111229841,0.458927795481119,-0.848045021297493));
#134966=DIRECTION('ref_axis',(-0.427750712273125,0.732266960571309,0.529919264233234));
#134967=DIRECTION('center_axis',(0.264962078570521,-0.458927782163207,0.848045038708646));
#134968=DIRECTION('ref_axis',(2.63879185457581E-16,-0.879478631391249,-0.475938375135033));
#134969=DIRECTION('center_axis',(-0.250002595299953,0.433017176051205,-0.866022417485787));
#134970=DIRECTION('ref_axis',(-0.436945896712322,0.747715375892674,0.499999999999942));
#134971=DIRECTION('center_axis',(-0.432988827019173,0.750027562856349,-0.499979330205085));
#134972=DIRECTION('ref_axis',(-0.249154705660435,0.433476564268119,0.866036951219501));
#134973=DIRECTION('center_axis',(-0.865904130412325,-0.500209992837883,
-3.49294771099265E-15));
#134974=DIRECTION('ref_axis',(-0.500209992837883,0.865904130412325,6.82961998416073E-15));
#134975=DIRECTION('center_axis',(0.500000000000004,-0.866025403784436,-5.97701461910994E-15));
#134976=DIRECTION('ref_axis',(-0.866025403784436,-0.500000000000004,-3.41480999208033E-15));
#134977=DIRECTION('center_axis',(-0.500000000000022,0.866025403784426,6.04742307255483E-15));
#134978=DIRECTION('ref_axis',(0.866025403784426,0.500000000000022,3.41480999208042E-15));
#134979=DIRECTION('center_axis',(-2.11225360334866E-16,-6.86101165903726E-15,
1.));
#134980=DIRECTION('ref_axis',(-1.,1.60344088833289E-30,-2.11560228140819E-16));
#134981=DIRECTION('center_axis',(-0.866146626230631,-0.499789977759954,
-3.49001476137941E-15));
#134982=DIRECTION('ref_axis',(-0.499789977759954,0.866146626230631,6.82961998416062E-15));
#134983=DIRECTION('center_axis',(-0.264962338412801,0.458928232223198,0.848044713969323));
#134984=DIRECTION('ref_axis',(-1.17907827621235E-15,-0.879478359737748,
0.475938877118691));
#134985=DIRECTION('center_axis',(-0.264962078570535,0.458927782163217,-0.848045038708636));
#134986=DIRECTION('ref_axis',(2.54209381385958E-16,0.879478631391243,0.475938375135045));
#134987=DIRECTION('center_axis',(-0.264962332887377,0.458928273073164,0.848044693589296));
#134988=DIRECTION('ref_axis',(0.427943903629752,-0.73215407445476,0.529919264233169));
#134989=DIRECTION('center_axis',(-0.264962371077225,0.458928288799655,0.848044673146737));
#134990=DIRECTION('ref_axis',(8.29844606197542E-17,-0.879478325588509,0.475938940222412));
#134991=DIRECTION('center_axis',(0.264962111362087,-0.458927795587544,0.848045021198581));
#134992=DIRECTION('ref_axis',(-0.420286434088522,0.736576463590586,0.52991926423328));
#134993=DIRECTION('center_axis',(-0.264962106632899,0.458927830768658,-0.848045003637561));
#134994=DIRECTION('ref_axis',(2.40514549107199E-15,0.879478602053312,0.475938429348116));
#134995=DIRECTION('center_axis',(-0.865896284857136,-0.500223573885327,
-7.16876759590109E-15));
#134996=DIRECTION('ref_axis',(-0.500223573885327,0.865896284857136,6.82961998416072E-15));
#134997=DIRECTION('center_axis',(-0.50000000000001,0.866025403784433,-7.61181689576648E-15));
#134998=DIRECTION('ref_axis',(0.866025403784433,0.50000000000001,3.41480999208034E-15));
#134999=DIRECTION('center_axis',(-2.11225360334866E-16,-6.86101165903726E-15,
1.));
#135000=DIRECTION('ref_axis',(-1.,1.70692667996567E-30,-2.10200002026934E-16));
#135001=DIRECTION('center_axis',(-0.866154464985103,-0.499776392786184,
2.38163428202604E-14));
#135002=DIRECTION('ref_axis',(-0.499776392786184,0.866154464985103,6.82961998416098E-15));
#135003=DIRECTION('center_axis',(-0.500000000000004,0.866025403784436,5.97701461910994E-15));
#135004=DIRECTION('ref_axis',(0.866025403784436,0.500000000000004,3.4148099920803E-15));
#135005=DIRECTION('center_axis',(-0.43303512883018,0.74997876016208,0.500012436350116));
#135006=DIRECTION('ref_axis',(0.249149002218687,-0.433518133176716,0.866017784401919));
#135007=DIRECTION('center_axis',(0.264962371077208,-0.458928288799654,-0.848044673146743));
#135008=DIRECTION('ref_axis',(-3.50114051472713E-16,0.879478325588511,-0.475938940222409));
#135009=DIRECTION('center_axis',(0.250002496045881,-0.433017045386664,-0.866022511471516));
#135010=DIRECTION('ref_axis',(0.42913023185866,-0.752228186194135,0.500000000000015));
#135011=DIRECTION('center_axis',(-0.250002511507148,0.433017051950186,0.866022503726369));
#135012=DIRECTION('ref_axis',(-1.26959939242869E-15,-0.894424794863834,
0.447218387740026));
#135013=DIRECTION('center_axis',(0.26496233271549,-0.458928272948179,-0.848044693710637));
#135014=DIRECTION('ref_axis',(0.420092076158679,-0.736687329158891,0.529919264233176));
#135015=DIRECTION('center_axis',(0.264962338412815,-0.458928232223186,-0.848044713969325));
#135016=DIRECTION('ref_axis',(3.76176649168549E-16,0.879478359737753,-0.475938877118681));
#135017=DIRECTION('center_axis',(-0.50000000000001,0.866025403784433,5.33644183083698E-14));
#135018=DIRECTION('ref_axis',(0.866025403784433,0.50000000000001,3.41480999208034E-15));
#135019=DIRECTION('center_axis',(0.50000000000001,-0.866025403784433,-6.04742307255487E-15));
#135020=DIRECTION('ref_axis',(-0.866025403784433,-0.50000000000001,-3.41480999208034E-15));
#135021=DIRECTION('center_axis',(-0.500000000000004,0.866025403784436,5.97701461910994E-15));
#135022=DIRECTION('ref_axis',(0.866025403784436,0.500000000000004,3.4148099920803E-15));
#135023=DIRECTION('center_axis',(-0.50000000000001,0.866025403784433,1.41659133449149E-13));
#135024=DIRECTION('ref_axis',(0.866025403784433,0.50000000000001,3.41480999208033E-15));
#135025=DIRECTION('center_axis',(-0.500000000000004,0.866025403784436,5.97701461910994E-15));
#135026=DIRECTION('ref_axis',(0.866025403784436,0.500000000000004,3.4148099920803E-15));
#135027=DIRECTION('center_axis',(0.433048509461644,-0.749993105181733,0.49997933020567));
#135028=DIRECTION('ref_axis',(0.250824363776384,-0.432512586706094,-0.866036951219159));
#135029=DIRECTION('center_axis',(-0.250002579266721,0.433017169313221,-0.866022425483285));
#135030=DIRECTION('ref_axis',(-5.6317795126628E-16,0.894424730216414,0.447218517033111));
#135031=DIRECTION('center_axis',(-0.25000258375266,0.433017177083137,-0.866022420303277));
#135032=DIRECTION('ref_axis',(-0.86602540378567,-0.499999999997868,1.38122234231956E-12));
#135033=DIRECTION('center_axis',(0.293895573516245,-0.40451255389424,-0.866022508719904));
#135034=DIRECTION('ref_axis',(0.809016994374529,0.587785252293049,-3.93386111998895E-13));
#135035=DIRECTION('center_axis',(0.509008435041564,-0.700641118228579,-0.500012436349281));
#135036=DIRECTION('ref_axis',(-0.294700492544349,0.403936649479602,-0.86601778440244));
#135037=DIRECTION('center_axis',(-0.293895578600006,0.404512560891461,0.866022503726318));
#135038=DIRECTION('ref_axis',(-1.11508461107079E-15,-0.906035256115486,
0.423202214875756));
#135039=DIRECTION('center_axis',(-0.58778525229247,0.80901699437495,5.6493354773342E-15));
#135040=DIRECTION('ref_axis',(0.80901699437495,0.58778525229247,3.41480999208022E-15));
#135041=DIRECTION('center_axis',(0.587785252292477,-0.809016994374945,-5.56656537619083E-15));
#135042=DIRECTION('ref_axis',(-0.809016994374945,-0.587785252292477,-3.41480999208033E-15));
#135043=DIRECTION('center_axis',(0.587785252292496,-0.809016994374931,-5.64933547733406E-15));
#135044=DIRECTION('ref_axis',(-0.809016994374931,-0.587785252292496,-3.41480999208037E-15));
#135045=DIRECTION('center_axis',(0.587785252292477,-0.809016994374945,-5.56656537619083E-15));
#135046=DIRECTION('ref_axis',(-0.809016994374945,-0.587785252292477,-3.41480999208033E-15));
#135047=DIRECTION('center_axis',(-0.58778525229247,0.80901699437495,5.6493354773342E-15));
#135048=DIRECTION('ref_axis',(0.80901699437495,0.58778525229247,3.41480999208022E-15));
#135049=DIRECTION('center_axis',(0.311481637390311,-0.428717694262762,0.848045003637585));
#135050=DIRECTION('ref_axis',(-4.68396541467905E-16,-0.89244205802627,-0.451162025292285));
#135051=DIRECTION('center_axis',(-0.293895658256084,0.404512670528685,-0.866022425483298));
#135052=DIRECTION('ref_axis',(-1.37831840766723E-15,0.906035197473495,0.423202340422599));
#135053=DIRECTION('center_axis',(-0.311481638273913,0.428717658687788,-0.84804502129749));
#135054=DIRECTION('ref_axis',(-0.501950189201556,0.683543400930059,0.529919264233232));
#135055=DIRECTION('center_axis',(0.311481604401037,-0.428717648856923,0.848045038708646));
#135056=DIRECTION('ref_axis',(4.76842727666993E-16,-0.892442084777734,-0.451161972375301));
#135057=DIRECTION('center_axis',(-0.293895674905427,0.404512675554181,-0.866022417485761));
#135058=DIRECTION('ref_axis',(-0.512709800571862,0.697946029716874,0.500000000000014));
#135059=DIRECTION('center_axis',(-0.509016097474244,0.70065917668986,-0.499979330205139));
#135060=DIRECTION('ref_axis',(-0.293100449232004,0.405058175800086,0.866036951219464));
#135061=DIRECTION('center_axis',(-0.808874435122379,-0.587981418248444,
-4.10585229880193E-15));
#135062=DIRECTION('ref_axis',(-0.587981418248444,0.808874435122379,6.82961998416087E-15));
#135063=DIRECTION('center_axis',(0.587785252292477,-0.809016994374945,-5.56656537619083E-15));
#135064=DIRECTION('ref_axis',(-0.809016994374945,-0.587785252292477,-3.41480999208033E-15));
#135065=DIRECTION('center_axis',(-0.58778525229247,0.80901699437495,5.6493354773342E-15));
#135066=DIRECTION('ref_axis',(0.80901699437495,0.58778525229247,3.41480999208022E-15));
#135067=DIRECTION('center_axis',(-2.23587008033243E-16,-6.86903940691702E-15,
1.));
#135068=DIRECTION('ref_axis',(-1.,1.60344088833289E-30,-2.25664243350207E-16));
#135069=DIRECTION('center_axis',(-0.809159506053914,-0.587589051772227,
-4.10311241834253E-15));
#135070=DIRECTION('ref_axis',(-0.587589051772227,0.809159506053914,6.82961998416088E-15));
#135071=DIRECTION('center_axis',(-0.311481909863919,0.428718069290538,0.848044713969328));
#135072=DIRECTION('ref_axis',(-3.03126833680443E-15,-0.892441837073397,
0.45116246235814));
#135073=DIRECTION('center_axis',(-0.311481604401053,0.428717648856944,-0.848045038708629));
#135074=DIRECTION('ref_axis',(5.0971935593662E-16,0.892442084777722,0.451161972375325));
#135075=DIRECTION('center_axis',(-0.311481908636353,0.428718110496056,0.848044693589286));
#135076=DIRECTION('ref_axis',(0.502130522416782,-0.683410939224696,0.529919264233211));
#135077=DIRECTION('center_axis',(-0.31148194826326,0.428718122142697,0.848044673146741));
#135078=DIRECTION('ref_axis',(3.18320034982604E-16,-0.892441805934779,0.451162523953254));
#135079=DIRECTION('center_axis',(0.311481638422179,-0.428717658775754,0.848045021198563));
#135080=DIRECTION('ref_axis',(-0.494977266831898,0.688609525576092,0.529919264233236));
#135081=DIRECTION('center_axis',(-0.311481637390301,0.428717694262749,-0.848045003637595));
#135082=DIRECTION('ref_axis',(-1.11423082982692E-15,0.892442058026277,0.45116202529227));
#135083=DIRECTION('center_axis',(-0.808865212939984,-0.587994104813606,
-4.10594088861296E-15));
#135084=DIRECTION('ref_axis',(-0.587994104813606,0.808865212939984,6.82961998416048E-15));
#135085=DIRECTION('center_axis',(-0.587785252292496,0.809016994374931,5.64933547733406E-15));
#135086=DIRECTION('ref_axis',(0.809016994374931,0.587785252292496,3.41480999208037E-15));
#135087=DIRECTION('center_axis',(-2.23587008033243E-16,-6.86903940691702E-15,
1.));
#135088=DIRECTION('ref_axis',(-1.,1.70692667996567E-30,-2.25214287886E-16));
#135089=DIRECTION('center_axis',(-0.80916872188328,-0.587576360591353,2.80003622398218E-14));
#135090=DIRECTION('ref_axis',(-0.587576360591353,0.809168721883279,6.82961998416027E-15));
#135091=DIRECTION('center_axis',(-0.587785252292477,0.809016994374945,5.56656537619083E-15));
#135092=DIRECTION('ref_axis',(0.809016994374945,0.587785252292477,3.41480999208025E-15));
#135093=DIRECTION('center_axis',(-0.509057044367654,0.700605801485977,0.500012436349198));
#135094=DIRECTION('ref_axis',(0.293099122184579,-0.40510011314894,0.86601778440246));
#135095=DIRECTION('center_axis',(0.311481948263274,-0.428718122142706,-0.848044673146732));
#135096=DIRECTION('ref_axis',(8.47741889849977E-16,0.892441805934773,-0.451162523953265));
#135097=DIRECTION('center_axis',(0.29389556253521,-0.404512555981462,-0.866022511471531));
#135098=DIRECTION('ref_axis',(0.505408667886012,-0.703251077799154,0.500000000000015));
#135099=DIRECTION('center_axis',(-0.293895578599989,0.40451256089141,0.866022503726348));
#135100=DIRECTION('ref_axis',(1.46405018279522E-15,-0.906035256115512,0.423202214875701));
#135101=DIRECTION('center_axis',(0.311481908456066,-0.428718110387007,-0.848044693710633));
#135102=DIRECTION('ref_axis',(0.494795562239831,-0.688740099734527,0.529919264233188));
#135103=DIRECTION('center_axis',(0.311481909863932,-0.428718069290516,-0.848044713969334));
#135104=DIRECTION('ref_axis',(1.60825548672769E-15,0.892441837073407,-0.45116246235812));
#135105=DIRECTION('center_axis',(-0.587785252292496,0.809016994374931,8.19663637794157E-14));
#135106=DIRECTION('ref_axis',(0.809016994374931,0.587785252292496,3.41480999208037E-15));
#135107=DIRECTION('center_axis',(0.587785252292496,-0.809016994374931,-5.64933547733406E-15));
#135108=DIRECTION('ref_axis',(-0.809016994374931,-0.587785252292496,-3.41480999208037E-15));
#135109=DIRECTION('center_axis',(-0.587785252292477,0.809016994374945,5.56656537619083E-15));
#135110=DIRECTION('ref_axis',(0.809016994374945,0.587785252292477,3.41480999208025E-15));
#135111=DIRECTION('center_axis',(-0.587785252292496,0.809016994374931,5.64933547733406E-15));
#135112=DIRECTION('ref_axis',(0.809016994374931,0.587785252292496,3.41480999208037E-15));
#135113=DIRECTION('center_axis',(-0.587785252292477,0.809016994374945,5.56656537619083E-15));
#135114=DIRECTION('ref_axis',(0.809016994374945,0.587785252292477,3.41480999208025E-15));
#135115=DIRECTION('center_axis',(0.509071851162528,-0.700618669263996,0.499979330205464));
#135116=DIRECTION('ref_axis',(0.294660197709419,-0.40392495219865,-0.866036951219268));
#135117=DIRECTION('center_axis',(-0.293895658256125,0.404512670528687,-0.866022425483283));
#135118=DIRECTION('ref_axis',(-1.31874420873521E-15,0.906035197473491,0.423202340422608));
#135119=DIRECTION('center_axis',(-0.293895663531681,0.404512677789842,-0.866022420301325));
#135120=DIRECTION('ref_axis',(-0.809016994375559,-0.587785252291632,6.29417776249093E-13));
#135121=DIRECTION('center_axis',(0.334568658444718,-0.371576139138295,-0.866022508719941));
#135122=DIRECTION('ref_axis',(0.743144825481234,0.669130606354594,3.34378195195858E-12));
#135123=DIRECTION('center_axis',(0.579456972966719,-0.643597063368448,-0.500012436349093));
#135124=DIRECTION('ref_axis',(-0.33530896966219,0.37091925261791,-0.866017784402521));
#135125=DIRECTION('center_axis',(-0.334568664232084,0.371576145565846,0.866022503726311));
#135126=DIRECTION('ref_axis',(-6.66659759826789E-17,-0.918982183096515,
0.394299058014553));
#135127=DIRECTION('center_axis',(-0.669130606358875,0.743144825477379,5.18935258042421E-15));
#135128=DIRECTION('ref_axis',(0.743144825477379,0.669130606358875,3.41480999208015E-15));
#135129=DIRECTION('center_axis',(0.669130606358862,-0.743144825477391,-5.09512767813147E-15));
#135130=DIRECTION('ref_axis',(-0.743144825477391,-0.669130606358862,-3.41480999208033E-15));
#135131=DIRECTION('center_axis',(0.669130606358845,-0.743144825477406,-3.77047027500057E-14));
#135132=DIRECTION('ref_axis',(-0.743144825477406,-0.669130606358845,-3.41480999208033E-15));
#135133=DIRECTION('center_axis',(0.669130606358862,-0.743144825477391,-5.09512767813147E-15));
#135134=DIRECTION('ref_axis',(-0.743144825477391,-0.669130606358862,-3.41480999208033E-15));
#135135=DIRECTION('center_axis',(-0.669130606358872,0.743144825477382,5.18935258042423E-15));
#135136=DIRECTION('ref_axis',(0.743144825477382,0.669130606358872,3.41480999208052E-15));
#135137=DIRECTION('center_axis',(0.354588510146763,-0.393810436983653,0.848045003637568));
#135138=DIRECTION('ref_axis',(2.80320064824192E-15,-0.906978223357755,-0.421177518814584));
#135139=DIRECTION('center_axis',(-0.334568754912021,0.371576246276131,-0.86602242548329));
#135140=DIRECTION('ref_axis',(2.58413282129854E-15,0.91898213146364,0.39429917835388));
#135141=DIRECTION('center_axis',(-0.354588507309677,0.393810401508679,-0.848045021297495));
#135142=DIRECTION('ref_axis',(-0.570650194820549,0.627330796745847,0.529919264233231));
#135143=DIRECTION('center_axis',(0.354588472592004,-0.393810395274868,0.84804503870863));
#135144=DIRECTION('ref_axis',(1.40544149701058E-15,-0.906978247051282,-0.421177467792122));
#135145=DIRECTION('center_axis',(-0.334568771995868,0.37157624953337,-0.866022417485767));
#135146=DIRECTION('ref_axis',(-0.582856348576968,0.640529840775232,0.49999999999998));
#135147=DIRECTION('center_axis',(-0.57946648104675,0.643614221961317,-0.499979330205185));
#135148=DIRECTION('ref_axis',(-0.333834922946612,0.372201885196443,0.866036951219429));
#135149=DIRECTION('center_axis',(-0.742982542253438,-0.669310796197565,
-4.67377230962008E-15));
#135150=DIRECTION('ref_axis',(-0.669310796197565,0.742982542253438,6.82961998416081E-15));
#135151=DIRECTION('center_axis',(0.669130606358862,-0.743144825477391,-5.09512767813147E-15));
#135152=DIRECTION('ref_axis',(-0.743144825477391,-0.669130606358862,-3.41480999208033E-15));
#135153=DIRECTION('center_axis',(-0.669130606358869,0.743144825477384,5.18935258042425E-15));
#135154=DIRECTION('ref_axis',(0.743144825477384,0.669130606358869,3.41480999208049E-15));
#135155=DIRECTION('center_axis',(-2.35041809182736E-16,-6.8783153219913E-15,
1.));
#135156=DIRECTION('ref_axis',(-1.,1.60344088833289E-30,-2.32716250954901E-16));
#135157=DIRECTION('center_axis',(-0.743307065001301,-0.668950377172442,
-4.67125551701931E-15));
#135158=DIRECTION('ref_axis',(-0.668950377172442,0.743307065001301,6.82961998416084E-15));
#135159=DIRECTION('center_axis',(-0.35458882032882,0.393810781475678,0.848044713969335));
#135160=DIRECTION('ref_axis',(8.82527612096891E-17,-0.906978027661855,0.421177940232642));
#135161=DIRECTION('center_axis',(-0.354588472592003,0.393810395274867,-0.848045038708631));
#135162=DIRECTION('ref_axis',(-1.80259659354061E-15,0.906978247051282,0.421177467792121));
#135163=DIRECTION('center_axis',(-0.354588823415871,0.393810822583094,0.848044693589303));
#135164=DIRECTION('ref_axis',(0.570815694129367,-0.627180210729071,0.529919264233191));
#135165=DIRECTION('center_axis',(-0.354588864042336,0.393810830024526,0.848044673146739));
#135166=DIRECTION('ref_axis',(-7.39505541680538E-17,-0.906978000082647,
0.421177999622584));
#135167=DIRECTION('center_axis',(0.354588507468212,-0.393810401579006,0.848045021198549));
#135168=DIRECTION('ref_axis',(-0.564245025055622,0.633098037506472,0.52991926423318));
#135169=DIRECTION('center_axis',(-0.354588510146757,0.393810436983647,-0.848045003637574));
#135170=DIRECTION('ref_axis',(-3.65482701585664E-15,0.906978223357759,0.421177518814577));
#135171=DIRECTION('center_axis',(-0.742972044483925,-0.669322449283883,
-4.67385368268692E-15));
#135172=DIRECTION('ref_axis',(-0.669322449283883,0.742972044483925,6.82961998416059E-15));
#135173=DIRECTION('center_axis',(-0.669130606358845,0.743144825477406,5.1893525804244E-15));
#135174=DIRECTION('ref_axis',(0.743144825477406,0.669130606358845,3.41480999208033E-15));
#135175=DIRECTION('center_axis',(-2.35041809182736E-16,-6.8783153219913E-15,
1.));
#135176=DIRECTION('ref_axis',(-1.,1.70692667996567E-30,-2.32721430815534E-16));
#135177=DIRECTION('center_axis',(-0.743317556935059,-0.668938718831625,
-4.6711741072605E-15));
#135178=DIRECTION('ref_axis',(-0.668938718831625,0.743317556935059,6.82961998416081E-15));
#135179=DIRECTION('center_axis',(-0.669130606358862,0.743144825477391,5.09512767813147E-15));
#135180=DIRECTION('ref_axis',(0.743144825477391,0.669130606358862,3.41480999208025E-15));
#135181=DIRECTION('center_axis',(-0.579501624401052,0.643556859035853,0.500012436349787));
#135182=DIRECTION('ref_axis',(0.333837986823119,-0.372243731516236,0.866017784402119));
#135183=DIRECTION('center_axis',(0.354588864042412,-0.393810830024448,-0.848044673146744));
#135184=DIRECTION('ref_axis',(3.48152255375756E-15,0.90697800008268,-0.421177999622512));
#135185=DIRECTION('center_axis',(0.334568647739284,-0.371576142364415,-0.866022511471548));
#135186=DIRECTION('ref_axis',(0.576149740768964,-0.646569003441916,0.499999999999983));
#135187=DIRECTION('center_axis',(-0.334568664232057,0.371576145565816,0.866022503726334));
#135188=DIRECTION('ref_axis',(2.06791103391257E-15,-0.91898218309653,0.394299058014518));
#135189=DIRECTION('center_axis',(0.354588823232584,-0.393810822486946,-0.848044693710589));
#135190=DIRECTION('ref_axis',(0.564077964606995,-0.633246889640457,0.529919264233257));
#135191=DIRECTION('center_axis',(0.354588820328813,-0.393810781475708,-0.848044713969324));
#135192=DIRECTION('ref_axis',(1.92894670706085E-15,0.906978027661841,-0.421177940232672));
#135193=DIRECTION('center_axis',(-0.669130606358845,0.743144825477406,-3.13699095091902E-14));
#135194=DIRECTION('ref_axis',(0.743144825477406,0.669130606358845,3.41480999208033E-15));
#135195=DIRECTION('center_axis',(0.669130606358875,-0.743144825477379,-5.18935258042421E-15));
#135196=DIRECTION('ref_axis',(-0.743144825477379,-0.669130606358875,-3.41480999208015E-15));
#135197=DIRECTION('center_axis',(-0.669130606358862,0.743144825477391,5.09512767813147E-15));
#135198=DIRECTION('ref_axis',(0.743144825477391,0.669130606358862,3.41480999208025E-15));
#135199=DIRECTION('center_axis',(-0.669130606358845,0.743144825477406,1.1454406603911E-15));
#135200=DIRECTION('ref_axis',(0.743144825477406,0.669130606358845,3.41480999208033E-15));
#135201=DIRECTION('center_axis',(-0.669130606358862,0.743144825477391,5.09512767813147E-15));
#135202=DIRECTION('ref_axis',(0.743144825477391,0.669130606358862,3.41480999208025E-15));
#135203=DIRECTION('center_axis',(0.579517695132059,-0.643568108591841,0.499979330205107));
#135204=DIRECTION('ref_axis',(0.335267672834652,-0.370911831402689,-0.866036951219485));
#135205=DIRECTION('center_axis',(-0.334568754912014,0.371576246276123,-0.866022425483296));
#135206=DIRECTION('ref_axis',(1.52738427012904E-15,0.918982131463644,0.394299178353872));
#135207=DIRECTION('center_axis',(-0.334568760917208,0.37157625294558,-0.866022420301719));
#135208=DIRECTION('ref_axis',(-0.743144825476697,-0.669130606359632,-6.3378873303023E-13));
#135209=DIRECTION('center_axis',(0.371576139132289,-0.334568658439294,-0.866022508724614));
#135210=DIRECTION('ref_axis',(0.66913060635532,0.74314482548058,-2.74058991357447E-12));
#135211=DIRECTION('center_axis',(0.643556859036948,-0.579501624401494,-0.500012436347864));
#135212=DIRECTION('ref_axis',(-0.372243731486086,0.33383798685376,-0.866017784403267));
#135213=DIRECTION('center_axis',(-0.371576145565853,0.334568664232079,0.86602250372631));
#135214=DIRECTION('ref_axis',(-0.918982183096512,-4.36450986441448E-16,
-0.39429905801456));
#135215=DIRECTION('center_axis',(-0.743144825477406,0.669130606358845,4.1231776140316E-14));
#135216=DIRECTION('ref_axis',(0.669130606358845,0.743144825477406,6.82961998416065E-15));
#135217=DIRECTION('center_axis',(0.743144825477398,-0.669130606358854,-4.56786669500649E-15));
#135218=DIRECTION('ref_axis',(-0.669130606358854,-0.743144825477398,-6.82961998416066E-15));
#135219=DIRECTION('center_axis',(0.743144825477406,-0.669130606358845,-4.6725140507014E-15));
#135220=DIRECTION('ref_axis',(-0.669130606358845,-0.743144825477406,-6.82961998416065E-15));
#135221=DIRECTION('center_axis',(0.743144825477398,-0.669130606358854,-4.56786669500649E-15));
#135222=DIRECTION('ref_axis',(-0.669130606358854,-0.743144825477398,-6.82961998416066E-15));
#135223=DIRECTION('center_axis',(-0.743144825477382,0.669130606358872,4.67251405070159E-15));
#135224=DIRECTION('ref_axis',(0.669130606358872,0.743144825477382,6.82961998416048E-15));
#135225=DIRECTION('center_axis',(0.393810436983641,-0.354588510146763,0.848045003637574));
#135226=DIRECTION('ref_axis',(-0.906978223357763,-4.0628693106624E-15,0.421177518814569));
#135227=DIRECTION('center_axis',(-0.371576246276136,0.334568754912025,-0.866022425483286));
#135228=DIRECTION('ref_axis',(0.918982131463637,2.78402616629794E-15,-0.394299178353887));
#135229=DIRECTION('center_axis',(-0.393810430455843,0.354588475160546,-0.848045021297515));
#135230=DIRECTION('ref_axis',(-0.63309803750285,0.564245025059696,0.529919264233169));
#135231=DIRECTION('center_axis',(0.393810395274834,-0.354588472591985,0.848045038708654));
#135232=DIRECTION('ref_axis',(-0.906978247051301,-4.04367791047371E-15,
0.42117746779208));
#135233=DIRECTION('center_axis',(-0.371576263602274,0.334568756370825,-0.866022417485744));
#135234=DIRECTION('ref_axis',(-0.646617000432134,0.576095872882387,0.500000000000031));
#135235=DIRECTION('center_axis',(-0.643568108591837,0.57951769513197,-0.499979330205214));
#135236=DIRECTION('ref_axis',(-0.370911831402169,0.335267672835389,0.866036951219422));
#135237=DIRECTION('center_axis',(-0.668950377172403,-0.743307065001336,
-5.19048549296485E-15));
#135238=DIRECTION('ref_axis',(-0.743307065001336,0.668950377172402,3.41480999208038E-15));
#135239=DIRECTION('center_axis',(0.743144825477398,-0.669130606358854,-4.56786669500649E-15));
#135240=DIRECTION('ref_axis',(-0.669130606358854,-0.743144825477398,-6.82961998416066E-15));
#135241=DIRECTION('center_axis',(-0.743144825477382,0.669130606358872,4.67251405070159E-15));
#135242=DIRECTION('ref_axis',(0.669130606358872,0.743144825477382,6.82961998416048E-15));
#135243=DIRECTION('center_axis',(-2.4546426258488E-16,-6.88873777539344E-15,
1.));
#135244=DIRECTION('ref_axis',(-1.,1.60344088833289E-30,-2.46820266164289E-16));
#135245=DIRECTION('center_axis',(-0.669310796197597,-0.742982542253409,
-5.18821936272801E-15));
#135246=DIRECTION('ref_axis',(-0.742982542253409,0.669310796197597,3.41480999208022E-15));
#135247=DIRECTION('center_axis',(-0.393810781475716,0.354588820328864,0.848044713969299));
#135248=DIRECTION('ref_axis',(-0.906978027661834,-3.05546561312248E-15,
-0.421177940232689));
#135249=DIRECTION('center_axis',(-0.393810395274935,0.354588472592013,-0.848045038708595));
#135250=DIRECTION('ref_axis',(0.906978247051249,3.61387669870221E-15,-0.421177467792193));
#135251=DIRECTION('center_axis',(-0.393810788844785,0.354588860886062,0.848044693589302));
#135252=DIRECTION('ref_axis',(0.633246889663017,-0.56407796458175,0.52991926423317));
#135253=DIRECTION('center_axis',(-0.393810830024481,0.354588864042376,0.848044673146743));
#135254=DIRECTION('ref_axis',(-0.906978000082666,2.6591822289014E-15,-0.421177999622544));
#135255=DIRECTION('center_axis',(0.393810430615192,-0.354588475220231,0.848045021198562));
#135256=DIRECTION('ref_axis',(-0.627330796754254,0.570650194811281,0.529919264233261));
#135257=DIRECTION('center_axis',(-0.393810436983659,0.35458851014678,-0.848045003637558));
#135258=DIRECTION('ref_axis',(0.906978223357751,-2.42657603144517E-15,-0.421177518814594));
#135259=DIRECTION('center_axis',(-0.668938718831589,-0.743317556935091,
-5.19055875774668E-15));
#135260=DIRECTION('ref_axis',(-0.743317556935091,0.668938718831589,3.41480999208028E-15));
#135261=DIRECTION('center_axis',(-0.743144825477406,0.669130606358845,4.6725140507014E-15));
#135262=DIRECTION('ref_axis',(0.669130606358845,0.743144825477406,6.82961998416065E-15));
#135263=DIRECTION('center_axis',(-2.4546426258488E-16,-6.88873777539344E-15,
1.));
#135264=DIRECTION('ref_axis',(-1.,1.70692667996567E-30,-2.477357166746E-16));
#135265=DIRECTION('center_axis',(-0.669322449283883,-0.742972044483925,
-5.18814605719551E-15));
#135266=DIRECTION('ref_axis',(-0.742972044483925,0.669322449283883,3.41480999208044E-15));
#135267=DIRECTION('center_axis',(-0.743144825477398,0.669130606358854,4.56786669500649E-15));
#135268=DIRECTION('ref_axis',(0.669130606358854,0.743144825477398,6.82961998416059E-15));
#135269=DIRECTION('center_axis',(-0.643597063368553,0.579456972966944,0.500012436348699));
#135270=DIRECTION('ref_axis',(0.370919252626752,-0.335308969651789,0.866017784402761));
#135271=DIRECTION('center_axis',(0.393810830024549,-0.354588864042312,-0.848044673146739));
#135272=DIRECTION('ref_axis',(0.906978000082638,1.23065481155338E-15,0.421177999622604));
#135273=DIRECTION('center_axis',(0.371576128830121,-0.334568662770661,-0.86602251147154));
#135274=DIRECTION('ref_axis',(0.64057839653263,-0.582802983773845,0.499999999999988));
#135275=DIRECTION('center_axis',(-0.371576145565821,0.33456866423205,0.866022503726335));
#135276=DIRECTION('ref_axis',(-0.918982183096528,1.60618320049483E-15,-0.394299058014522));
#135277=DIRECTION('center_axis',(0.393810788644162,-0.354588860818729,-0.84804469371062));
#135278=DIRECTION('ref_axis',(0.627180210740024,-0.570815694117288,0.529919264233239));
#135279=DIRECTION('center_axis',(0.39381078147571,-0.354588820328811,-0.848044713969325));
#135280=DIRECTION('ref_axis',(0.906978027661841,2.25474419065798E-15,0.421177940232673));
#135281=DIRECTION('center_axis',(-0.743144825477406,0.669130606358845,4.6725140507014E-15));
#135282=DIRECTION('ref_axis',(0.669130606358845,0.743144825477406,6.82961998416065E-15));
#135283=DIRECTION('center_axis',(0.743144825477406,-0.669130606358845,-4.6725140507014E-15));
#135284=DIRECTION('ref_axis',(-0.669130606358845,-0.743144825477406,-6.82961998416065E-15));
#135285=DIRECTION('center_axis',(-0.743144825477398,0.669130606358854,4.56786669500649E-15));
#135286=DIRECTION('ref_axis',(0.669130606358854,0.743144825477398,6.82961998416059E-15));
#135287=DIRECTION('center_axis',(-0.743144825477406,0.669130606358845,4.6725140507014E-15));
#135288=DIRECTION('ref_axis',(0.669130606358845,0.743144825477406,6.82961998416065E-15));
#135289=DIRECTION('center_axis',(-0.743144825477398,0.669130606358854,4.56786669500649E-15));
#135290=DIRECTION('ref_axis',(0.669130606358854,0.743144825477398,6.82961998416059E-15));
#135291=DIRECTION('center_axis',(0.643614221961007,-0.579466481046877,0.499979330205437));
#135292=DIRECTION('ref_axis',(0.372201885211874,-0.333834922929833,-0.866036951219265));
#135293=DIRECTION('center_axis',(-0.371576246276125,0.334568754912027,-0.86602242548329));
#135294=DIRECTION('ref_axis',(0.918982131463642,2.65789370359083E-15,-0.394299178353875));
#135295=DIRECTION('center_axis',(-0.371576252946193,0.334568760917773,-0.866022420301237));
#135296=DIRECTION('ref_axis',(-0.669130606358731,-0.743144825477509,-8.30481788101122E-14));
#135297=DIRECTION('center_axis',(0.404512553891932,-0.293895573514563,-0.866022508721553));
#135298=DIRECTION('ref_axis',(0.587785252287783,0.809016994378355,-3.36126577915125E-12));
#135299=DIRECTION('center_axis',(0.700605801485285,-0.509057044368013,-0.500012436349802));
#135300=DIRECTION('ref_axis',(-0.405100113137893,0.293099122200829,-0.866017784402128));
#135301=DIRECTION('center_axis',(-0.404512560891477,0.2938955786,0.866022503726312));
#135302=DIRECTION('ref_axis',(-0.906035256115478,-1.80341242297892E-15,
-0.423202214875772));
#135303=DIRECTION('center_axis',(-0.80901699437495,0.58778525229247,4.10448247925272E-15));
#135304=DIRECTION('ref_axis',(0.58778525229247,0.80901699437495,6.82961998416043E-15));
#135305=DIRECTION('center_axis',(0.809016994374951,-0.587785252292469,-3.99055920848346E-15));
#135306=DIRECTION('ref_axis',(-0.587785252292469,-0.80901699437495,-6.82961998416066E-15));
#135307=DIRECTION('center_axis',(0.80901699437495,-0.58778525229247,-4.10448247925272E-15));
#135308=DIRECTION('ref_axis',(-0.58778525229247,-0.80901699437495,-6.82961998416043E-15));
#135309=DIRECTION('center_axis',(0.809016994374951,-0.587785252292469,-3.99055920848346E-15));
#135310=DIRECTION('ref_axis',(-0.587785252292469,-0.80901699437495,-6.82961998416066E-15));
#135311=DIRECTION('center_axis',(-0.809016994374976,0.587785252292434,4.10448247925247E-15));
#135312=DIRECTION('ref_axis',(0.587785252292434,0.809016994374976,6.82961998416065E-15));
#135313=DIRECTION('center_axis',(0.428717694262762,-0.3114816373903,0.84804500363759));
#135314=DIRECTION('ref_axis',(-0.892442058026271,-6.18994737741828E-16,
0.451162025292283));
#135315=DIRECTION('center_axis',(-0.404512670528675,0.293895658256107,-0.866022425483295));
#135316=DIRECTION('ref_axis',(0.906035197473498,-1.65240743153779E-15,-0.423202340422593));
#135317=DIRECTION('center_axis',(-0.428717684113514,0.311481603278345,-0.848045021297511));
#135318=DIRECTION('ref_axis',(-0.68860952557912,0.494977266827708,0.529919264233214));
#135319=DIRECTION('center_axis',(0.428717648856936,-0.311481604401036,0.848045038708639));
#135320=DIRECTION('ref_axis',(-0.892442084777727,-6.11447499249856E-16,
0.451161972375315));
#135321=DIRECTION('center_axis',(-0.404512687918747,0.293895657887068,-0.866022417485759));
#135322=DIRECTION('ref_axis',(-0.70329318114634,0.505350078018259,0.500000000000001));
#135323=DIRECTION('center_axis',(-0.700618669263931,0.50907185116259,-0.499979330205492));
#135324=DIRECTION('ref_axis',(-0.403924952200305,0.294660197707191,0.866036951219254));
#135325=DIRECTION('center_axis',(-0.587589051772227,-0.809159506053914,
-5.65033063106954E-15));
#135326=DIRECTION('ref_axis',(-0.809159506053914,0.587589051772227,3.41480999208049E-15));
#135327=DIRECTION('center_axis',(0.809016994374951,-0.587785252292469,-3.99055920848346E-15));
#135328=DIRECTION('ref_axis',(-0.587785252292469,-0.80901699437495,-6.82961998416066E-15));
#135329=DIRECTION('center_axis',(-0.80901699437495,0.58778525229247,4.10448247925272E-15));
#135330=DIRECTION('ref_axis',(0.58778525229247,0.80901699437495,6.82961998416043E-15));
#135331=DIRECTION('center_axis',(-2.54740177659163E-16,-6.90019257654294E-15,
1.));
#135332=DIRECTION('ref_axis',(-1.,2.00430111041611E-30,-2.53872273768983E-16));
#135333=DIRECTION('center_axis',(-0.587981418248456,-0.808874435122371,
-5.64833999139408E-15));
#135334=DIRECTION('ref_axis',(-0.808874435122371,0.587981418248456,3.41480999208034E-15));
#135335=DIRECTION('center_axis',(-0.428718069290576,0.311481909863944,0.8480447139693));
#135336=DIRECTION('ref_axis',(-0.892441837073374,1.48661188715482E-15,-0.451162462358185));
#135337=DIRECTION('center_axis',(-0.428717648856939,0.311481604401038,-0.848045038708637));
#135338=DIRECTION('ref_axis',(0.892442084777726,5.36066018208771E-16,-0.451161972375317));
#135339=DIRECTION('center_axis',(-0.428718080856456,0.311481949431746,0.848044693589292));
#135340=DIRECTION('ref_axis',(0.688740099742912,-0.494795562228176,0.529919264233172));
#135341=DIRECTION('center_axis',(-0.428718122142682,0.311481948263276,0.848044673146743));
#135342=DIRECTION('ref_axis',(-0.892441805934786,1.06689281669451E-15,-0.451162523953241));
#135343=DIRECTION('center_axis',(0.428717684276344,-0.311481603323609,0.84804502119857));
#135344=DIRECTION('ref_axis',(-0.683543400924064,0.501950189209757,0.529919264233197));
#135345=DIRECTION('center_axis',(-0.428717694262774,0.311481637390308,-0.84804500363758));
#135346=DIRECTION('ref_axis',(0.892442058026264,1.61640809885533E-15,-0.451162025292297));
#135347=DIRECTION('center_axis',(-0.587576360591347,-0.809168721883284,
-4.98609139731183E-14));
#135348=DIRECTION('ref_axis',(-0.809168721883284,0.587576360591347,3.41480999207922E-15));
#135349=DIRECTION('center_axis',(-0.80901699437495,0.58778525229247,-4.0097746579219E-14));
#135350=DIRECTION('ref_axis',(0.58778525229247,0.80901699437495,6.82961998416043E-15));
#135351=DIRECTION('center_axis',(-2.54740177659163E-16,-6.90019257654294E-15,
1.));
#135352=DIRECTION('ref_axis',(-1.,1.70692667996567E-30,-2.55242859604134E-16));
#135353=DIRECTION('center_axis',(-0.587994104813612,-0.80886521293998,6.41945027862958E-15));
#135354=DIRECTION('ref_axis',(-0.80886521293998,0.587994104813612,3.41480999208017E-15));
#135355=DIRECTION('center_axis',(-0.809016994374951,0.587785252292469,3.99055920848346E-15));
#135356=DIRECTION('ref_axis',(0.587785252292469,0.809016994374951,6.82961998416065E-15));
#135357=DIRECTION('center_axis',(-0.700641118228681,0.509008435041422,0.500012436349283));
#135358=DIRECTION('ref_axis',(0.403936649448406,-0.294700492587247,0.866017784402393));
#135359=DIRECTION('center_axis',(0.428718122142701,-0.311481948263281,-0.848044673146731));
#135360=DIRECTION('ref_axis',(0.892441805934775,3.97758164497583E-16,0.451162523953261));
#135361=DIRECTION('center_axis',(0.404512544092706,-0.293895578898575,-0.866022511471566));
#135362=DIRECTION('ref_axis',(0.697988741328929,-0.512651652663007,0.499999999999945));
#135363=DIRECTION('center_axis',(-0.404512560891434,0.293895578599976,0.86602250372634));
#135364=DIRECTION('ref_axis',(-0.906035256115501,1.10927932520561E-15,-0.423202214875725));
#135365=DIRECTION('center_axis',(0.428718080653436,-0.311481949380818,-0.848044693710632));
#135366=DIRECTION('ref_axis',(0.683410939228537,-0.502130522411571,0.529919264233195));
#135367=DIRECTION('center_axis',(0.42871806929053,-0.311481909863932,-0.848044713969327));
#135368=DIRECTION('ref_axis',(0.8924418370734,2.85180820314112E-15,0.451162462358134));
#135369=DIRECTION('center_axis',(-0.80901699437495,0.58778525229247,4.10448247925272E-15));
#135370=DIRECTION('ref_axis',(0.58778525229247,0.80901699437495,6.82961998416043E-15));
#135371=DIRECTION('center_axis',(0.809016994374976,-0.587785252292434,-4.10448247925247E-15));
#135372=DIRECTION('ref_axis',(-0.587785252292434,-0.809016994374976,-6.82961998416065E-15));
#135373=DIRECTION('center_axis',(-0.809016994374951,0.587785252292469,3.99055920848346E-15));
#135374=DIRECTION('ref_axis',(0.587785252292469,0.809016994374951,6.82961998416065E-15));
#135375=DIRECTION('center_axis',(-0.80901699437495,0.58778525229247,3.62192817228647E-14));
#135376=DIRECTION('ref_axis',(0.58778525229247,0.80901699437495,6.82961998416044E-15));
#135377=DIRECTION('center_axis',(-0.809016994374951,0.587785252292469,3.99055920848346E-15));
#135378=DIRECTION('ref_axis',(0.587785252292469,0.809016994374951,6.82961998416065E-15));
#135379=DIRECTION('center_axis',(0.700659176689191,-0.509016097474679,0.499979330205633));
#135380=DIRECTION('ref_axis',(0.405058175807095,-0.29310044922319,-0.866036951219169));
#135381=DIRECTION('center_axis',(-0.404512670528692,0.293895658256119,-0.866022425483283));
#135382=DIRECTION('ref_axis',(0.906035197473489,-1.02813875008142E-16,-0.423202340422611));
#135383=DIRECTION('center_axis',(-0.404512677788109,0.293895663530384,-0.866022420302574));
#135384=DIRECTION('ref_axis',(-0.587785252290296,-0.809016994376529,-1.56043157028568E-12));
#135385=DIRECTION('center_axis',(0.433017044463491,-0.250002507184682,-0.866022508717571));
#135386=DIRECTION('ref_axis',(0.500000000006304,0.866025403780799,4.21797331194789E-12));
#135387=DIRECTION('center_axis',(0.749978760165048,-0.433035128827861,-0.500012436347673));
#135388=DIRECTION('ref_axis',(-0.433518133167728,0.249149002229375,-0.866017784403343));
#135389=DIRECTION('center_axis',(-0.433017051950273,0.250002511507189,0.866022503726313));
#135390=DIRECTION('ref_axis',(-0.894424794863787,-3.51926008997178E-16,
-0.447218387740121));
#135391=DIRECTION('center_axis',(-0.86602540378444,0.499999999999998,6.44677165429795E-14));
#135392=DIRECTION('ref_axis',(0.499999999999998,0.86602540378444,6.82961998416156E-15));
#135393=DIRECTION('center_axis',(0.866025403784442,-0.499999999999995,-3.36953032019409E-15));
#135394=DIRECTION('ref_axis',(-0.499999999999995,-0.866025403784441,-6.82961998416066E-15));
#135395=DIRECTION('center_axis',(0.866025403784433,-0.50000000000001,-1.71507213071646E-14));
#135396=DIRECTION('ref_axis',(-0.50000000000001,-0.866025403784433,-6.82961998416068E-15));
#135397=DIRECTION('center_axis',(0.866025403784442,-0.499999999999995,-3.36953032019409E-15));
#135398=DIRECTION('ref_axis',(-0.499999999999995,-0.866025403784441,-6.82961998416066E-15));
#135399=DIRECTION('center_axis',(-0.86602540378444,0.499999999999998,3.49148133884312E-15));
#135400=DIRECTION('ref_axis',(0.499999999999998,0.86602540378444,6.82961998416073E-15));
#135401=DIRECTION('center_axis',(0.45892783076861,-0.264962106632881,0.848045003637592));
#135402=DIRECTION('ref_axis',(-0.87947860205334,1.19060858178351E-15,0.475938429348065));
#135403=DIRECTION('center_axis',(-0.43301716931323,0.250002579266689,-0.86602242548329));
#135404=DIRECTION('ref_axis',(0.894424730216411,1.60782206696907E-16,-0.447218517033116));
#135405=DIRECTION('center_axis',(-0.458927817107794,0.264962073771327,-0.848045021297498));
#135406=DIRECTION('ref_axis',(-0.736576463606657,0.420286434060449,0.529919264233207));
#135407=DIRECTION('center_axis',(0.45892778216319,-0.264962078570529,0.848045038708653));
#135408=DIRECTION('ref_axis',(-0.879478631391258,1.16952532199408E-15,0.475938375135017));
#135409=DIRECTION('center_axis',(-0.433017186567245,0.250002577085764,-0.866022417485751));
#135410=DIRECTION('ref_axis',(-0.752263934580233,0.42906756196414,0.500000000000016));
#135411=DIRECTION('center_axis',(-0.749993105181609,0.433048509462133,-0.499979330205433));
#135412=DIRECTION('ref_axis',(-0.432512586699257,0.250824363787739,0.866036951219285));
#135413=DIRECTION('center_axis',(-0.499789977759954,-0.866146626230631,
-6.04826956437238E-15));
#135414=DIRECTION('ref_axis',(-0.866146626230631,0.499789977759954,3.41480999208016E-15));
#135415=DIRECTION('center_axis',(0.866025403784442,-0.499999999999995,-3.36953032019409E-15));
#135416=DIRECTION('ref_axis',(-0.499999999999995,-0.866025403784441,-6.82961998416066E-15));
#135417=DIRECTION('center_axis',(-0.866025403784457,0.499999999999969,3.49148133884292E-15));
#135418=DIRECTION('ref_axis',(0.499999999999969,0.866025403784457,6.82961998416065E-15));
#135419=DIRECTION('center_axis',(-2.62767925538921E-16,-6.91255422424131E-15,
1.));
#135420=DIRECTION('ref_axis',(-1.,2.00430111041611E-30,-2.60924281373677E-16));
#135421=DIRECTION('center_axis',(-0.500209992837911,-0.865904130412309,
-6.04657622512354E-15));
#135422=DIRECTION('ref_axis',(-0.865904130412309,0.500209992837911,3.41480999208024E-15));
#135423=DIRECTION('center_axis',(-0.458928232223204,0.264962338412787,0.848044713969324));
#135424=DIRECTION('ref_axis',(-0.879478359737745,-9.91663607721953E-16,
-0.475938877118696));
#135425=DIRECTION('center_axis',(-0.45892778216322,0.264962078570537,-0.848045038708634));
#135426=DIRECTION('ref_axis',(0.879478631391241,1.07865946136944E-15,-0.475938375135048));
#135427=DIRECTION('center_axis',(-0.458928247863733,0.264962376551373,0.848044693589302));
#135428=DIRECTION('ref_axis',(0.736687329152564,-0.420092076169725,0.529919264233214));
#135429=DIRECTION('center_axis',(-0.458928288799617,0.264962371077277,0.848044673146741));
#135430=DIRECTION('ref_axis',(-0.879478325588526,2.57091442443615E-15,-0.475938940222381));
#135431=DIRECTION('center_axis',(0.458927817277461,-0.264962073794094,0.848045021198568));
#135432=DIRECTION('ref_axis',(-0.732266960570914,0.427750712273813,0.529919264233224));
#135433=DIRECTION('center_axis',(-0.458927830768617,0.264962106632877,-0.84804500363759));
#135434=DIRECTION('ref_axis',(0.879478602053337,-8.27701491930472E-16,-0.475938429348071));
#135435=DIRECTION('center_axis',(-0.499776392786171,-0.866154464985111,
-6.04832430210234E-15));
#135436=DIRECTION('ref_axis',(-0.86615446498511,0.499776392786171,3.41480999208032E-15));
#135437=DIRECTION('center_axis',(-0.866025403784433,0.50000000000001,1.71507213071653E-14));
#135438=DIRECTION('ref_axis',(0.50000000000001,0.866025403784433,6.82961998416068E-15));
#135439=DIRECTION('center_axis',(-2.62767925538921E-16,-6.91255422424131E-15,
1.));
#135440=DIRECTION('ref_axis',(-1.,1.70692667996567E-30,-2.62750002533667E-16));
#135441=DIRECTION('center_axis',(-0.500223573885299,-0.865896284857153,
-9.72224648886353E-15));
#135442=DIRECTION('ref_axis',(-0.865896284857153,0.500223573885299,3.41480999208028E-15));
#135443=DIRECTION('center_axis',(-0.866025403784442,0.499999999999995,3.36953032019409E-15));
#135444=DIRECTION('ref_axis',(0.499999999999995,0.866025403784442,6.82961998416074E-15));
#135445=DIRECTION('center_axis',(-0.750008802378862,0.432983094186076,0.500012436348614));
#135446=DIRECTION('ref_axis',(0.432528431874663,-0.250863215155224,0.866017784402854));
#135447=DIRECTION('center_axis',(0.458928288799688,-0.264962371077173,-0.848044673146735));
#135448=DIRECTION('ref_axis',(0.879478325588494,1.64057136930641E-15,0.475938940222439));
#135449=DIRECTION('center_axis',(0.433017035275494,-0.250002513558742,-0.866022511471574));
#135450=DIRECTION('ref_axis',(0.74775177542025,-0.436883602754709,0.499999999999929));
#135451=DIRECTION('center_axis',(-0.43301705195022,0.250002511507158,0.866022503726349));
#135452=DIRECTION('ref_axis',(-0.894424794863815,2.91747672552896E-15,-0.447218387740063));
#135453=DIRECTION('center_axis',(0.458928247653565,-0.264962376527061,-0.848044693710632));
#135454=DIRECTION('ref_axis',(0.732154074456122,-0.427943903627455,0.529919264233141));
#135455=DIRECTION('center_axis',(0.458928232223194,-0.264962338412781,-0.848044713969331));
#135456=DIRECTION('ref_axis',(0.879478359737751,1.00929923944428E-16,0.475938877118685));
#135457=DIRECTION('center_axis',(-0.866025403784433,0.50000000000001,3.4914813388432E-15));
#135458=DIRECTION('ref_axis',(0.50000000000001,0.866025403784433,6.82961998416068E-15));
#135459=DIRECTION('center_axis',(0.866025403784433,-0.50000000000001,-3.4914813388432E-15));
#135460=DIRECTION('ref_axis',(-0.50000000000001,-0.866025403784433,-6.82961998416068E-15));
#135461=DIRECTION('center_axis',(-0.866025403784442,0.499999999999995,3.36953032019409E-15));
#135462=DIRECTION('ref_axis',(0.499999999999995,0.866025403784442,6.82961998416074E-15));
#135463=DIRECTION('center_axis',(-0.866025403784433,0.50000000000001,3.4914813388432E-15));
#135464=DIRECTION('ref_axis',(0.50000000000001,0.866025403784433,6.82961998416068E-15));
#135465=DIRECTION('center_axis',(-0.866025403784442,0.499999999999995,3.36953032019409E-15));
#135466=DIRECTION('ref_axis',(0.499999999999995,0.866025403784442,6.82961998416074E-15));
#135467=DIRECTION('center_axis',(0.75002756285576,-0.432988827019632,0.499979330205573));
#135468=DIRECTION('ref_axis',(0.433476564276502,-0.249154705646875,-0.866036951219207));
#135469=DIRECTION('center_axis',(-0.433017169313196,0.250002579266716,-0.866022425483299));
#135470=DIRECTION('ref_axis',(0.894424730216427,-1.69509643524011E-15,-0.447218517033086));
#135471=DIRECTION('center_axis',(-0.433017177085375,0.250002583753999,-0.866022420301771));
#135472=DIRECTION('ref_axis',(-0.500000000003883,-0.866025403782197,2.5744935431098E-12));
#135473=DIRECTION('center_axis',(0.456777309669419,-0.203370361062852,-0.86602250872153));
#135474=DIRECTION('ref_axis',(0.406736643074989,0.913545457642962,-4.89547161595317E-13));
#135475=DIRECTION('center_axis',(0.791134794600545,-0.352268789801452,-0.500012436349511));
#135476=DIRECTION('ref_axis',(0.457186437800744,-0.202469153675368,0.866017784402287));
#135477=DIRECTION('center_axis',(-0.456777317573304,0.203370364581841,0.86602250372631));
#135478=DIRECTION('ref_axis',(-0.884507036382085,2.80052133003465E-16,-0.466526850878468));
#135479=DIRECTION('center_axis',(-0.913545457642594,0.406736643075817,2.84022679824583E-15));
#135480=DIRECTION('ref_axis',(0.406736643075817,0.913545457642593,6.82961998416057E-15));
#135481=DIRECTION('center_axis',(0.913545457642603,-0.406736643075795,-2.71158415259712E-15));
#135482=DIRECTION('ref_axis',(-0.406736643075795,-0.913545457642603,-6.82961998416066E-15));
#135483=DIRECTION('center_axis',(0.913545457642598,-0.406736643075807,-2.84022679824576E-15));
#135484=DIRECTION('ref_axis',(-0.406736643075807,-0.913545457642598,-6.8296199841606E-15));
#135485=DIRECTION('center_axis',(0.913545457642603,-0.406736643075795,-2.71158415259712E-15));
#135486=DIRECTION('ref_axis',(-0.406736643075795,-0.913545457642603,-6.82961998416066E-15));
#135487=DIRECTION('center_axis',(-0.913545457642603,0.406736643075797,2.84022679824569E-15));
#135488=DIRECTION('ref_axis',(0.406736643075797,0.913545457642603,6.82961998416064E-15));
#135489=DIRECTION('center_axis',(0.484109857923767,-0.215539595588311,0.848045003637577));
#135490=DIRECTION('ref_axis',(-0.868458021515997,-9.89659158812798E-17,
0.495762710240011));
#135491=DIRECTION('center_axis',(-0.456777441376074,0.203370419702476,-0.866022425483293));
#135492=DIRECTION('ref_axis',(0.884506966812058,1.8236239182919E-15,-0.466526982779059));
#135493=DIRECTION('center_axis',(-0.484109840902953,0.215539564334311,-0.84804502129751));
#135494=DIRECTION('ref_axis',(-0.776473315754038,0.340990855180143,0.529919264233189));
#135495=DIRECTION('center_axis',(0.484109806651284,-0.215539572760331,0.848045038708647));
#135496=DIRECTION('ref_axis',(-0.868458052949959,4.03183191579828E-16,0.495762655175201));
#135497=DIRECTION('center_axis',(-0.456777458307734,0.203370415729553,-0.86602241748578));
#135498=DIRECTION('ref_axis',(-0.792992726925484,0.34808409191359,0.499999999999977));
#135499=DIRECTION('center_axis',(-0.791150459692779,0.352280597670813,-0.499979330205359));
#135500=DIRECTION('ref_axis',(0.456361522796281,-0.204240445636448,-0.866036951219337));
#135501=DIRECTION('center_axis',(-0.406515100163568,-0.913644062717536,
-6.3799423906462E-15));
#135502=DIRECTION('ref_axis',(-0.913644062717536,0.406515100163568,3.41480999208032E-15));
#135503=DIRECTION('center_axis',(0.913545457642603,-0.406736643075795,-2.71158415259712E-15));
#135504=DIRECTION('ref_axis',(-0.406736643075795,-0.913545457642603,-6.82961998416066E-15));
#135505=DIRECTION('center_axis',(-0.913545457642603,0.406736643075797,2.84022679824569E-15));
#135506=DIRECTION('ref_axis',(0.406736643075797,0.913545457642603,6.82961998416064E-15));
#135507=DIRECTION('center_axis',(-2.6945955253847E-16,-6.92568728168955E-15,
1.));
#135508=DIRECTION('ref_axis',(-1.,2.00430111041611E-30,-2.67976288978371E-16));
#135509=DIRECTION('center_axis',(-0.406958162070199,-0.913446798847336,
-6.37856490440294E-15));
#135510=DIRECTION('ref_axis',(-0.913446798847336,0.406958162070199,3.4148099920803E-15));
#135511=DIRECTION('center_axis',(-0.484110281406756,0.21553978413508,0.848044713969301));
#135512=DIRECTION('ref_axis',(-0.868457761888264,-2.62723474582901E-16,
-0.495763165045597));
#135513=DIRECTION('center_axis',(-0.484109806651301,0.215539572760338,-0.848045038708636));
#135514=DIRECTION('ref_axis',(0.868458052949949,2.96622001727381E-16,-0.495762655175219));
#135515=DIRECTION('center_axis',(-0.48411030094316,0.2155398204412,0.848044693589258));
#135516=DIRECTION('ref_axis',(0.776563258046704,-0.340785973371052,0.529919264233178));
#135517=DIRECTION('center_axis',(-0.484110341087582,0.215539810706753,0.848044673146741));
#135518=DIRECTION('ref_axis',(-0.868457725299283,2.05000090583624E-15,-0.495763229140681));
#135519=DIRECTION('center_axis',(0.484109841073579,-0.215539564340363,0.848045021198569));
#135520=DIRECTION('ref_axis',(-0.772967650155533,0.348864709031412,0.529919264233206));
#135521=DIRECTION('center_axis',(-0.484109857923745,0.215539595588301,-0.848045003637592));
#135522=DIRECTION('ref_axis',(0.86845802151601,-1.31527569561181E-15,-0.495762710239987));
#135523=DIRECTION('center_axis',(-0.406500770236713,-0.913650438514074,
-6.37998691259547E-15));
#135524=DIRECTION('ref_axis',(-0.913650438514073,0.406500770236713,3.41480999208024E-15));
#135525=DIRECTION('center_axis',(-0.913545457642598,0.406736643075807,2.84022679824576E-15));
#135526=DIRECTION('ref_axis',(0.406736643075807,0.913545457642598,6.82961998416061E-15));
#135527=DIRECTION('center_axis',(-2.6945955253847E-16,-6.92568728168955E-15,
1.));
#135528=DIRECTION('ref_axis',(-1.,2.13365834995709E-30,-2.70257145463201E-16));
#135529=DIRECTION('center_axis',(-0.406972488803014,-0.913440415876964,
-6.37852033235906E-15));
#135530=DIRECTION('ref_axis',(-0.913440415876964,0.406972488803014,3.41480999208024E-15));
#135531=DIRECTION('center_axis',(-0.913545457642603,0.406736643075795,2.71158415259712E-15));
#135532=DIRECTION('ref_axis',(0.406736643075795,0.913545457642603,6.82961998416064E-15));
#135533=DIRECTION('center_axis',(-0.791159233140825,0.352213899939985,0.500012436350425));
#135534=DIRECTION('ref_axis',(0.456381342217505,-0.204277427964079,0.866017784401757));
#135535=DIRECTION('center_axis',(0.484110341087604,-0.215539810706705,-0.84804467314674));
#135536=DIRECTION('ref_axis',(0.868457725299273,-1.11516049819258E-15,0.495763229140698));
#135537=DIRECTION('center_axis',(0.456777301206547,-0.203370368360254,-0.866022511471542));
#135538=DIRECTION('ref_axis',(0.7893222845842,-0.356328964664343,0.500000000000017));
#135539=DIRECTION('center_axis',(-0.456777317573169,0.20337036458186,0.866022503726376));
#135540=DIRECTION('ref_axis',(-0.884507036382157,1.69032347061982E-15,-0.466526850878333));
#135541=DIRECTION('center_axis',(0.484110300737792,-0.215539820425012,-0.848044693710607));
#135542=DIRECTION('ref_axis',(0.772875576442627,-0.349068641864353,0.529919264233197));
#135543=DIRECTION('center_axis',(0.484110281406739,-0.215539784135015,-0.848044713969328));
#135544=DIRECTION('ref_axis',(0.868457761888278,-1.33747047041045E-15,0.495763165045573));
#135545=DIRECTION('center_axis',(-0.913545457642598,0.406736643075807,2.84022679824576E-15));
#135546=DIRECTION('ref_axis',(0.406736643075807,0.913545457642598,6.82961998416061E-15));
#135547=DIRECTION('center_axis',(0.913545457642598,-0.406736643075807,-2.84022679824576E-15));
#135548=DIRECTION('ref_axis',(-0.406736643075807,-0.913545457642598,-6.8296199841606E-15));
#135549=DIRECTION('center_axis',(-0.913545457642603,0.406736643075795,2.71158415259712E-15));
#135550=DIRECTION('ref_axis',(0.406736643075795,0.913545457642603,6.82961998416064E-15));
#135551=DIRECTION('center_axis',(-0.913545457642598,0.406736643075807,-8.27120002511786E-15));
#135552=DIRECTION('ref_axis',(0.406736643075807,0.913545457642598,6.8296199841606E-15));
#135553=DIRECTION('center_axis',(-0.913545457642603,0.406736643075795,2.71158415259712E-15));
#135554=DIRECTION('ref_axis',(0.406736643075795,0.913545457642603,6.82961998416064E-15));
#135555=DIRECTION('center_axis',(0.791178490090583,-0.352217640366738,0.499979330205232));
#135556=DIRECTION('ref_axis',(0.457145692799107,-0.202479170972784,-0.866036951219403));
#135557=DIRECTION('center_axis',(-0.456777441376052,0.203370419702467,-0.866022425483307));
#135558=DIRECTION('ref_axis',(0.88450696681207,8.66756486764032E-16,-0.466526982779037));
#135559=DIRECTION('center_axis',(-0.456777449573532,0.203370423352227,-0.866022420302521));
#135560=DIRECTION('ref_axis',(-0.406736643075106,-0.91354545764291,-4.45837591507382E-13));
#135561=DIRECTION('center_axis',(0.475533027095179,-0.15451004671247,-0.866022508718224));
#135562=DIRECTION('ref_axis',(0.309016994378645,0.951056516293952,2.26852657916475E-12));
#135563=DIRECTION('center_axis',(0.82362299067401,-0.267642920194133,-0.500012436348495));
#135564=DIRECTION('ref_axis',(0.475845712146801,-0.153571010706525,0.866017784402884));
#135565=DIRECTION('center_axis',(-0.475533035318161,0.154510049384242,0.866022503726304));
#135566=DIRECTION('ref_axis',(-0.876548788012425,1.94488523957394E-15,-0.481313018974086));
#135567=DIRECTION('center_axis',(-0.951056516295146,0.309016994374972,2.15785413849121E-15));
#135568=DIRECTION('ref_axis',(0.309016994374972,0.951056516295146,6.82961998416073E-15));
#135569=DIRECTION('center_axis',(0.951056516295156,-0.309016994374942,-2.02392930158883E-15));
#135570=DIRECTION('ref_axis',(-0.309016994374942,-0.951056516295155,-6.82961998416066E-15));
#135571=DIRECTION('center_axis',(0.951056516295148,-0.309016994374964,1.47258949833367E-14));
#135572=DIRECTION('ref_axis',(-0.309016994374964,-0.951056516295148,-6.82961998416061E-15));
#135573=DIRECTION('center_axis',(0.951056516295156,-0.309016994374942,-2.02392930158883E-15));
#135574=DIRECTION('ref_axis',(-0.309016994374942,-0.951056516295155,-6.82961998416066E-15));
#135575=DIRECTION('center_axis',(-0.951056516295146,0.309016994374972,2.15785413849121E-15));
#135576=DIRECTION('ref_axis',(0.309016994374972,0.951056516295146,6.82961998416073E-15));
#135577=DIRECTION('center_axis',(0.503987876168977,-0.163755587629907,0.848045003637583));
#135578=DIRECTION('ref_axis',(-0.859649462041492,4.39826809004255E-16,0.510884333691857));
#135579=DIRECTION('center_axis',(-0.475533164204401,0.154510091261986,-0.866022425483291));
#135580=DIRECTION('ref_axis',(0.876548714628841,4.29963435206314E-16,-0.481313152617427));
#135581=DIRECTION('center_axis',(-0.503987855972783,0.163755558331625,-0.848045021297487));
#135582=DIRECTION('ref_axis',(-0.807862963765476,0.257959309137282,0.529919264233221));
#135583=DIRECTION('center_axis',(0.503987822791196,-0.163755570286415,0.848045038708653));
#135584=DIRECTION('ref_axis',(-0.859649495083707,2.20200626090829E-15,0.510884278092727));
#135585=DIRECTION('center_axis',(-0.475533180627341,0.154510085543092,-0.866022417485778));
#135586=DIRECTION('ref_axis',(-0.825033325010143,0.263286939711698,0.499999999999955));
#135587=DIRECTION('center_axis',(-0.823639804208689,0.267653025932082,-0.499979330205232));
#135588=DIRECTION('ref_axis',(0.475210466541726,-0.155418826439376,-0.866036951219405));
#135589=DIRECTION('center_axis',(-0.308786358060986,-0.951131423661017,
-6.64171523299948E-15));
#135590=DIRECTION('ref_axis',(-0.951131423661017,0.308786358060986,3.41480999208039E-15));
#135591=DIRECTION('center_axis',(0.951056516295156,-0.309016994374942,-2.02392930158883E-15));
#135592=DIRECTION('ref_axis',(-0.309016994374942,-0.951056516295155,-6.82961998416066E-15));
#135593=DIRECTION('center_axis',(-0.951056516295162,0.309016994374922,2.15785413849087E-15));
#135594=DIRECTION('ref_axis',(0.309016994374922,0.951056516295162,6.82961998416065E-15));
#135595=DIRECTION('center_axis',(-2.74741743792088E-16,-6.93944786036197E-15,
1.));
#135596=DIRECTION('ref_axis',(-1.,2.00430111041611E-30,-2.75028296583065E-16));
#135597=DIRECTION('center_axis',(-0.309247612517378,-0.95098155300316,-6.64066869178919E-15));
#135598=DIRECTION('ref_axis',(-0.95098155300316,0.309247612517378,3.41480999208029E-15));
#135599=DIRECTION('center_axis',(-0.503988317040574,0.163755730877717,0.848044713969325));
#135600=DIRECTION('ref_axis',(-0.859649189130472,-2.17897991428701E-16,
-0.510884792910615));
#135601=DIRECTION('center_axis',(-0.503987822791213,0.16375557028642,-0.848045038708642));
#135602=DIRECTION('ref_axis',(0.859649495083697,-1.26799831889259E-15,-0.510884278092745));
#135603=DIRECTION('center_axis',(-0.503988340268016,0.163755764933399,0.848044693589299));
#135604=DIRECTION('ref_axis',(0.807930997358871,-0.257746148179274,0.529919264233193));
#135605=DIRECTION('center_axis',(-0.503988379172003,0.163755751065505,0.848044673146734));
#135606=DIRECTION('ref_axis',(-0.859649150669465,2.12951299205037E-15,-0.510884857627693));
#135607=DIRECTION('center_axis',(0.503987856146397,-0.163755558309613,0.84804502119856));
#135608=DIRECTION('ref_axis',(-0.80519954441769,0.26615647101673,0.529919264233209));
#135609=DIRECTION('center_axis',(-0.503987876169011,0.163755587629918,-0.84804500363756));
#135610=DIRECTION('ref_axis',(0.859649462041471,1.57485748646909E-15,-0.510884333691893));
#135611=DIRECTION('center_axis',(-0.308771440182777,-0.951136266645034,
-6.64174905137613E-15));
#135612=DIRECTION('ref_axis',(-0.951136266645034,0.308771440182777,3.41480999208035E-15));
#135613=DIRECTION('center_axis',(-0.951056516295148,0.309016994374964,-4.98049825795553E-14));
#135614=DIRECTION('ref_axis',(0.309016994374964,0.951056516295148,6.82961998416031E-15));
#135615=DIRECTION('center_axis',(-2.74741743792088E-16,-6.93944786036197E-15,
1.));
#135616=DIRECTION('ref_axis',(-1.,2.13365834995709E-30,-2.77764288392734E-16));
#135617=DIRECTION('center_axis',(-0.309262527968948,-0.950976702550728,
2.44143881663588E-15));
#135618=DIRECTION('ref_axis',(-0.950976702550728,0.309262527968948,3.41480999208024E-15));
#135619=DIRECTION('center_axis',(-0.951056516295156,0.309016994374942,2.02392930158883E-15));
#135620=DIRECTION('ref_axis',(0.309016994374942,0.951056516295156,6.8296199841606E-15));
#135621=DIRECTION('center_axis',(-0.823641557783644,0.267585776504662,0.500012436349466));
#135622=DIRECTION('ref_axis',(0.475234043100657,-0.155453534463189,0.866017784402321));
#135623=DIRECTION('center_axis',(0.503988379172001,-0.163755751065456,-0.848044673146744));
#135624=DIRECTION('ref_axis',(0.859649150669468,-2.26336925852521E-15,0.510884857627687));
#135625=DIRECTION('center_axis',(0.475533019434099,-0.154510054858537,-0.866022511471556));
#135626=DIRECTION('ref_axis',(0.822244813610406,-0.271870311896699,0.499999999999979));
#135627=DIRECTION('center_axis',(-0.475533035318099,0.154510049384272,0.866022503726332));
#135628=DIRECTION('ref_axis',(-0.876548788012458,8.76596332424742E-17,-0.481313018974026));
#135629=DIRECTION('center_axis',(0.503988340058683,-0.163755764949449,-0.848044693710605));
#135630=DIRECTION('ref_axis',(0.805129291878303,-0.266368911012672,0.529919264233209));
#135631=DIRECTION('center_axis',(0.503988317040564,-0.163755730877724,-0.84804471396933));
#135632=DIRECTION('ref_axis',(0.859649189130478,-1.64241712406884E-16,0.510884792910606));
#135633=DIRECTION('center_axis',(-0.951056516295148,0.309016994374964,-4.98049825795553E-14));
#135634=DIRECTION('ref_axis',(0.309016994374964,0.951056516295148,6.82961998416031E-15));
#135635=DIRECTION('center_axis',(0.951056516295165,-0.309016994374914,-2.15785413849081E-15));
#135636=DIRECTION('ref_axis',(-0.309016994374914,-0.951056516295164,-6.82961998416067E-15));
#135637=DIRECTION('center_axis',(-0.951056516295156,0.309016994374942,2.02392930158883E-15));
#135638=DIRECTION('ref_axis',(0.309016994374942,0.951056516295156,6.8296199841606E-15));
#135639=DIRECTION('center_axis',(-0.951056516295148,0.309016994374964,-4.98049825795525E-14));
#135640=DIRECTION('ref_axis',(0.309016994374964,0.951056516295148,6.82961998416031E-15));
#135641=DIRECTION('center_axis',(-0.951056516295156,0.309016994374942,2.02392930158883E-15));
#135642=DIRECTION('ref_axis',(0.309016994374942,0.951056516295156,6.8296199841606E-15));
#135643=DIRECTION('center_axis',(0.823661100222817,-0.267587483540044,0.499979330205204));
#135644=DIRECTION('ref_axis',(0.475806237451048,-0.153585232119715,-0.86603695121941));
#135645=DIRECTION('center_axis',(-0.475533164204424,0.154510091261989,-0.866022425483278));
#135646=DIRECTION('ref_axis',(0.876548714628828,1.33063653772379E-15,-0.48131315261745));
#135647=DIRECTION('center_axis',(-0.475533172741877,0.154510094035947,-0.866022420300449));
#135648=DIRECTION('ref_axis',(-0.309016994382379,-0.951056516292739,4.51956930993777E-12));
#135649=DIRECTION('center_axis',(0.489078705150955,-0.103956887952906,-0.866022508723077));
#135650=DIRECTION('ref_axis',(0.207911690818348,0.978147600733681,3.58418457596544E-13));
#135651=DIRECTION('center_axis',(0.847087400906921,-0.180084698747046,-0.50001243634728));
#135652=DIRECTION('ref_axis',(0.489291521297257,-0.102990311599294,0.866017784403586));
#135653=DIRECTION('center_axis',(-0.48907871361637,0.103956889752263,0.866022503726313));
#135654=DIRECTION('ref_axis',(-0.870740345484703,9.01293367321942E-17,-0.491743073916837));
#135655=DIRECTION('center_axis',(-0.978147600733807,0.207911690817751,1.45183957723501E-15));
#135656=DIRECTION('ref_axis',(0.207911690817752,0.978147600733807,6.82961998416061E-15));
#135657=DIRECTION('center_axis',(0.978147600733807,-0.207911690817753,-1.3140998576179E-15));
#135658=DIRECTION('ref_axis',(-0.207911690817753,-0.978147600733807,-6.82961998416066E-15));
#135659=DIRECTION('center_axis',(0.978147600733806,-0.207911690817757,-4.29175525433417E-15));
#135660=DIRECTION('ref_axis',(-0.207911690817757,-0.978147600733806,-6.8296199841607E-15));
#135661=DIRECTION('center_axis',(0.978147600733807,-0.207911690817753,-1.3140998576179E-15));
#135662=DIRECTION('ref_axis',(-0.207911690817753,-0.978147600733807,-6.82961998416066E-15));
#135663=DIRECTION('center_axis',(-0.978147600733807,0.207911690817751,1.45183957723501E-15));
#135664=DIRECTION('ref_axis',(0.207911690817752,0.978147600733807,6.82961998416061E-15));
#135665=DIRECTION('center_axis',(0.518344097776653,-0.11017743918536,0.848045003637581));
#135666=DIRECTION('ref_axis',(-0.853239582811868,-1.49305978118172E-15,
0.521519140898039));
#135667=DIRECTION('center_axis',(-0.489078846173993,0.103956917928318,-0.86602242548329));
#135668=DIRECTION('ref_axis',(0.87074026939378,-1.88754034186863E-16,-0.491743208652694));
#135669=DIRECTION('center_axis',(-0.518344074628652,0.110177412158262,-0.848045021297499));
#135670=DIRECTION('ref_axis',(-0.830401496087922,0.172101506935423,0.52991926423324));
#135671=DIRECTION('center_axis',(0.518344042878396,-0.110177427516375,0.848045038708649));
#135672=DIRECTION('ref_axis',(-0.853239616987304,-4.00876318608133E-16,
0.521519084984776));
#135673=DIRECTION('center_axis',(-0.489078861910606,0.103956910517348,-0.86602241748578));
#135674=DIRECTION('ref_axis',(-0.848034685338871,0.175605160693646,0.499999999999961));
#135675=DIRECTION('center_axis',(-0.847105178671992,0.180092991630944,-0.499979330205268));
#135676=DIRECTION('ref_axis',(0.488852904975874,-0.104894406043765,-0.866036951219389));
#135677=DIRECTION('center_axis',(-0.207674488001825,-0.978197989689807,
6.5307210243107E-15));
#135678=DIRECTION('ref_axis',(-0.978197989689807,0.207674488001825,7.66186706172843E-29));
#135679=DIRECTION('center_axis',(0.978147600733807,-0.207911690817753,-1.3140998576179E-15));
#135680=DIRECTION('ref_axis',(-0.207911690817753,-0.978147600733807,-6.82961998416066E-15));
#135681=DIRECTION('center_axis',(-0.978147600733807,0.207911690817751,1.45183957723501E-15));
#135682=DIRECTION('ref_axis',(0.207911690817751,0.978147600733807,6.82961998416071E-15));
#135683=DIRECTION('center_axis',(-2.78556626507032E-16,-6.95368519647906E-15,
1.));
#135684=DIRECTION('ref_axis',(-1.,2.00430111041611E-30,-2.75028296583065E-16));
#135685=DIRECTION('center_axis',(-0.208148881407613,-0.978097154258594,
-6.83001592333891E-15));
#135686=DIRECTION('ref_axis',(-0.978097154258594,0.208148881407613,-1.2419109941013E-29));
#135687=DIRECTION('center_axis',(-0.518344551206596,0.110177535564887,0.848044713969305));
#135688=DIRECTION('ref_axis',(-0.853239300541031,5.99666814548819E-16,-0.521519602711396));
#135689=DIRECTION('center_axis',(-0.518344042878388,0.110177427516373,-0.848045038708654));
#135690=DIRECTION('ref_axis',(0.853239616987309,3.25739190337144E-16,-0.521519084984768));
#135691=DIRECTION('center_axis',(-0.518344577867247,0.1101775670028,0.8480446935893));
#135692=DIRECTION('ref_axis',(0.830446875603153,-0.171882402227476,0.529919264233216));
#135693=DIRECTION('center_axis',(-0.51834461510783,0.11017754914753,0.848044673146739));
#135694=DIRECTION('ref_axis',(-0.853239260760977,-1.33244400003472E-15,
-0.521519667794093));
#135695=DIRECTION('center_axis',(0.518344074797558,-0.110177412125059,0.848045021198573));
#135696=DIRECTION('ref_axis',(-0.828609503967322,0.18053216702172,0.529919264233213));
#135697=DIRECTION('center_axis',(-0.518344097776682,0.110177439185366,-0.848045003637562));
#135698=DIRECTION('ref_axis',(0.85323958281185,-6.83615864401498E-16,-0.521519140898069));
#135699=DIRECTION('center_axis',(-0.207659145615642,-0.978201246800566,
-4.81512163663705E-15));
#135700=DIRECTION('ref_axis',(-0.978201246800566,0.207659145615642,3.22797051853182E-29));
#135701=DIRECTION('center_axis',(-0.978147600733806,0.207911690817757,4.29175525433432E-15));
#135702=DIRECTION('ref_axis',(0.207911690817757,0.978147600733806,6.8296199841607E-15));
#135703=DIRECTION('center_axis',(-2.78556626507032E-16,-6.95368519647906E-15,
1.));
#135704=DIRECTION('ref_axis',(-1.,2.13365834995709E-30,-2.77764288392734E-16));
#135705=DIRECTION('center_axis',(-0.208164222161104,-0.978093889466682,
-6.82999312541884E-15));
#135706=DIRECTION('ref_axis',(-0.978093889466682,0.208164222161104,3.8857267529552E-29));
#135707=DIRECTION('center_axis',(-0.978147600733807,0.207911690817753,1.3140998576179E-15));
#135708=DIRECTION('ref_axis',(0.207911690817753,0.978147600733807,6.8296199841607E-15));
#135709=DIRECTION('center_axis',(-0.84709989316117,0.18002592730352,0.50001243635018));
#135710=DIRECTION('ref_axis',(0.488879980354404,-0.10492645952426,0.866017784401904));
#135711=DIRECTION('center_axis',(0.518344615107833,-0.110177549147486,-0.848044673146743));
#135712=DIRECTION('ref_axis',(0.853239260760977,1.13050245003069E-15,0.521519667794094));
#135713=DIRECTION('center_axis',(0.48907869839261,-0.103956896852029,-0.866022511471548));
#135714=DIRECTION('ref_axis',(0.846158656401662,-0.184432991074133,0.499999999999983));
#135715=DIRECTION('center_axis',(-0.489078713616272,0.103956889752265,0.866022503726369));
#135716=DIRECTION('ref_axis',(-0.870740345484759,1.36101104600592E-16,-0.491743073916738));
#135717=DIRECTION('center_axis',(0.518344577661257,-0.110177567038289,-0.848044693710595));
#135718=DIRECTION('ref_axis',(0.828561842309987,-0.180750786616231,0.529919264233236));
#135719=DIRECTION('center_axis',(0.518344551206575,-0.110177535564853,-0.848044713969322));
#135720=DIRECTION('ref_axis',(0.853239300541046,-1.38182160689371E-15,0.521519602711372));
#135721=DIRECTION('center_axis',(-0.978147600733806,0.207911690817757,1.45183957723504E-15));
#135722=DIRECTION('ref_axis',(0.207911690817757,0.978147600733806,6.8296199841607E-15));
#135723=DIRECTION('center_axis',(0.978147600733806,-0.20791169081776,-1.45183957723506E-15));
#135724=DIRECTION('ref_axis',(-0.20791169081776,-0.978147600733805,-6.82961998416069E-15));
#135725=DIRECTION('center_axis',(-0.978147600733807,0.207911690817753,1.3140998576179E-15));
#135726=DIRECTION('ref_axis',(0.207911690817753,0.978147600733807,6.8296199841607E-15));
#135727=DIRECTION('center_axis',(-0.978147600733806,0.207911690817757,1.45183957723504E-15));
#135728=DIRECTION('ref_axis',(0.207911690817757,0.978147600733806,6.8296199841607E-15));
#135729=DIRECTION('center_axis',(-0.978147600733807,0.207911690817753,1.3140998576179E-15));
#135730=DIRECTION('ref_axis',(0.207911690817753,0.978147600733807,6.8296199841607E-15));
#135731=DIRECTION('center_axis',(0.847119506978456,-0.180025582247714,0.499979330205709));
#135732=DIRECTION('ref_axis',(0.489253749392351,-0.103008581334865,-0.866036951219118));
#135733=DIRECTION('center_axis',(-0.489078846173999,0.103956917928292,-0.86602242548329));
#135734=DIRECTION('ref_axis',(0.870740269393778,5.30090735249655E-17,-0.491743208652699));
#135735=DIRECTION('center_axis',(-0.489078854953935,0.103956919794531,-0.866022420300872));
#135736=DIRECTION('ref_axis',(-0.207911690814671,-0.978147600734462,-1.82268897705632E-12));
#135737=DIRECTION('center_axis',(0.497265934580328,-0.0522647557777281,
-0.866022508719865));
#135738=DIRECTION('ref_axis',(0.104528463270788,0.994521895367944,1.84891472637859E-12));
#135739=DIRECTION('center_axis',(0.861270944309348,-0.0905534316548714,
-0.500012436349348));
#135740=DIRECTION('ref_axis',(0.497376550152134,-0.0512812290952578,0.8660177844024));
#135741=DIRECTION('center_axis',(-0.497265943181917,0.0522647566818097,
0.866022503726312));
#135742=DIRECTION('ref_axis',(-0.867207748104377,6.21980953328682E-15,-0.497946504785137));
#135743=DIRECTION('center_axis',(-0.994521895368276,0.104528463267628,7.29918357753749E-16));
#135744=DIRECTION('ref_axis',(0.104528463267628,0.994521895368276,6.82961998416064E-15));
#135745=DIRECTION('center_axis',(0.994521895368274,-0.104528463267647,-5.89872860613828E-16));
#135746=DIRECTION('ref_axis',(-0.104528463267647,-0.994521895368274,-6.82961998416066E-15));
#135747=DIRECTION('center_axis',(0.994521895368276,-0.104528463267629,-2.15769772104621E-15));
#135748=DIRECTION('ref_axis',(-0.104528463267629,-0.994521895368276,-6.82961998416064E-15));
#135749=DIRECTION('center_axis',(0.994521895368274,-0.104528463267647,-5.89872860613828E-16));
#135750=DIRECTION('ref_axis',(-0.104528463267647,-0.994521895368274,-6.82961998416066E-15));
#135751=DIRECTION('center_axis',(-0.994521895368276,0.104528463267627,7.29918357753739E-16));
#135752=DIRECTION('ref_axis',(0.104528463267627,0.994521895368276,6.82961998416064E-15));
#135753=DIRECTION('center_axis',(0.527021232978627,-0.0553921636609854,
0.848045003637568));
#135754=DIRECTION('ref_axis',(-0.849349030019368,-6.14256318298022E-15,
0.527831625809934));
#135755=DIRECTION('center_axis',(-0.497266077958573,0.0522647708473914,
-0.866022425483294));
#135756=DIRECTION('ref_axis',(0.867207670398082,6.7132432122382E-15,-0.497946640115918));
#135757=DIRECTION('center_axis',(-0.527021207132412,0.0553921392005488,
-0.848045021297503));
#135758=DIRECTION('ref_axis',(-0.843841975853136,0.0843581245808926,0.529919264233213));
#135759=DIRECTION('center_axis',(0.527021177161346,-0.0553921577943527,
0.848045038708649));
#135760=DIRECTION('ref_axis',(-0.84934906486752,-6.45825246295237E-15,0.527831569734768));
#135761=DIRECTION('center_axis',(-0.497266092833451,0.0522647618405224,
-0.866022417485776));
#135762=DIRECTION('ref_axis',(-0.861744800189367,0.0859994148039461,0.499999999999967));
#135763=DIRECTION('center_axis',(-0.86128949152969,0.0905598208269947,-0.49997933020507));
#135764=DIRECTION('ref_axis',(0.497139368681892,-0.0532207405904418,-0.866036951219505));
#135765=DIRECTION('center_axis',(-0.104287292793437,-0.994547213842468,
-1.52506548609107E-16));
#135766=DIRECTION('ref_axis',(-0.994547213842468,0.104287292793437,-1.21159629448723E-31));
#135767=DIRECTION('center_axis',(0.994521895368274,-0.104528463267647,-5.89872860613828E-16));
#135768=DIRECTION('ref_axis',(-0.104528463267647,-0.994521895368274,-6.82961998416066E-15));
#135769=DIRECTION('center_axis',(-0.994521895368276,0.104528463267628,7.29918357753744E-16));
#135770=DIRECTION('ref_axis',(0.104528463267628,0.994521895368276,6.82961998416064E-15));
#135771=DIRECTION('center_axis',(-2.80862404029962E-16,-6.96824330280696E-15,
1.));
#135772=DIRECTION('ref_axis',(-1.,2.00430111041611E-30,-2.82080304187759E-16));
#135773=DIRECTION('center_axis',(-0.104769627595152,-0.994496518411992,
-6.94453207115987E-15));
#135774=DIRECTION('ref_axis',(-0.994496518411992,0.104769627595152,1.55544708777506E-29));
#135775=DIRECTION('center_axis',(-0.527021693998977,0.0553922121162114,
0.848044713969329));
#135776=DIRECTION('ref_axis',(-0.849348742192414,6.03707679245365E-15,-0.527832088960271));
#135777=DIRECTION('center_axis',(-0.527021177161337,0.0553921577943518,
-0.848045038708655));
#135778=DIRECTION('ref_axis',(0.849349064867526,6.34435230052652E-15,-0.527831569734759));
#135779=DIRECTION('center_axis',(-0.527021723799262,0.0553922406001627,
0.848044693589287));
#135780=DIRECTION('ref_axis',(0.843864204097289,-0.0841354766899499,0.52991926423315));
#135781=DIRECTION('center_axis',(-0.527021758969971,0.055392218944938,0.848044673146736));
#135782=DIRECTION('ref_axis',(-0.849348701629311,6.94167645812496E-15,-0.527832154231442));
#135783=DIRECTION('center_axis',(0.527021207296535,-0.0553921391535296,
0.848045021198579));
#135784=DIRECTION('ref_axis',(-0.842941044395143,0.092929914820619,0.529919264233202));
#135785=DIRECTION('center_axis',(-0.527021232978637,0.0553921636609864,
-0.848045003637562));
#135786=DIRECTION('ref_axis',(0.849349030019363,6.26358979594039E-15,-0.527831625809943));
#135787=DIRECTION('center_axis',(-0.104271693993661,-0.994548849394384,
-5.84959516006002E-15));
#135788=DIRECTION('ref_axis',(-0.994548849394384,0.104271693993661,-2.64454906907446E-29));
#135789=DIRECTION('center_axis',(-0.994521895368276,0.104528463267629,7.29918357753754E-16));
#135790=DIRECTION('ref_axis',(0.104528463267629,0.994521895368276,6.82961998416064E-15));
#135791=DIRECTION('center_axis',(-2.80862404029962E-16,-6.96824330280696E-15,
1.));
#135792=DIRECTION('ref_axis',(-1.,2.13365834995709E-30,-2.77764288392734E-16));
#135793=DIRECTION('center_axis',(-0.104785225574079,-0.994494875050339,
-1.26696667606311E-14));
#135794=DIRECTION('ref_axis',(-0.994494875050339,0.104785225574079,1.43090320927726E-29));
#135795=DIRECTION('center_axis',(-0.994521895368274,0.104528463267647,5.89872860613828E-16));
#135796=DIRECTION('ref_axis',(0.104528463267647,0.994521895368274,6.82961998416068E-15));
#135797=DIRECTION('center_axis',(-0.861277224843024,0.090493676372023,0.500012436348713));
#135798=DIRECTION('ref_axis',(0.497169646239502,-0.053249788320922,0.86601778440276));
#135799=DIRECTION('center_axis',(0.527021758969985,-0.0553922189448753,
-0.848044673146731));
#135800=DIRECTION('ref_axis',(0.849348701629303,-6.77688496309739E-15,0.527832154231454));
#135801=DIRECTION('center_axis',(0.497265928783437,-0.0522647653361823,
-0.866022511471555));
#135802=DIRECTION('ref_axis',(0.860801807879653,-0.0949749838175252,0.499999999999983));
#135803=DIRECTION('center_axis',(-0.497265943181819,0.052264756681772,0.86602250372637));
#135804=DIRECTION('ref_axis',(-0.867207748104435,6.1483298530269E-15,-0.497946504785037));
#135805=DIRECTION('center_axis',(0.527021723597929,-0.0553922406581351,
-0.84804469371062));
#135806=DIRECTION('ref_axis',(0.84291649580075,-0.0931523188200768,0.529919264233173));
#135807=DIRECTION('center_axis',(0.527021693998996,-0.0553922121161665,
-0.84804471396932));
#135808=DIRECTION('ref_axis',(0.849348742192403,-7.26099966146184E-15,0.52783208896029));
#135809=DIRECTION('center_axis',(-0.994521895368276,0.104528463267629,7.29918357753754E-16));
#135810=DIRECTION('ref_axis',(0.104528463267629,0.994521895368276,6.82961998416064E-15));
#135811=DIRECTION('center_axis',(0.994521895368276,-0.104528463267628,-7.29918357753749E-16));
#135812=DIRECTION('ref_axis',(-0.104528463267628,-0.994521895368276,-6.82961998416064E-15));
#135813=DIRECTION('center_axis',(-0.994521895368274,0.104528463267647,5.89872860613828E-16));
#135814=DIRECTION('ref_axis',(0.104528463267647,0.994521895368274,6.82961998416068E-15));
#135815=DIRECTION('center_axis',(-0.994521895368276,0.104528463267629,5.5067571248093E-14));
#135816=DIRECTION('ref_axis',(0.104528463267629,0.994521895368276,6.8296199841606E-15));
#135817=DIRECTION('center_axis',(-0.994521895368274,0.104528463267647,5.89872860613828E-16));
#135818=DIRECTION('ref_axis',(0.104528463267647,0.994521895368274,6.82961998416068E-15));
#135819=DIRECTION('center_axis',(0.861296695145372,-0.0904912830026448,
0.499979330204954));
#135820=DIRECTION('ref_axis',(0.497340894868293,-0.0513033470048911,-0.866036951219578));
#135821=DIRECTION('center_axis',(-0.497266077958585,0.0522647708473931,
-0.866022425483287));
#135822=DIRECTION('ref_axis',(0.867207670398075,6.99786079247477E-15,-0.497946640115931));
#135823=DIRECTION('center_axis',(-0.497266086881794,0.052264771785269,-0.866022420303021));
#135824=DIRECTION('ref_axis',(-0.104528463266305,-0.994521895368415,-7.78030306748679E-13));
#135825=DIRECTION('center_axis',(0.500005014363881,6.27963960171735E-15,
-0.866022508720747));
#135826=DIRECTION('ref_axis',(3.35689482235833E-12,1.,1.94507577597585E-12));
#135827=DIRECTION('center_axis',(0.866018223014528,-3.00422161454986E-5,
-0.500012436349562));
#135828=DIRECTION('ref_axis',(0.50001221744103,0.000989701338965518,0.86601778440224));
#135829=DIRECTION('center_axis',(-0.500005023014372,-2.60454852281367E-14,
0.866022503726316));
#135830=DIRECTION('ref_axis',(-0.866022503726316,3.41480999208025E-15,-0.500005023014372));
#135831=DIRECTION('center_axis',(-1.,0.,0.));
#135832=DIRECTION('ref_axis',(0.,6.82961998416066E-15,-1.));
#135833=DIRECTION('center_axis',(1.,-9.83319205199467E-31,1.4081690688991E-16));
#135834=DIRECTION('ref_axis',(-1.4081690688991E-16,-6.82961998416066E-15,
1.));
#135835=DIRECTION('center_axis',(1.,0.,0.));
#135836=DIRECTION('ref_axis',(0.,-6.82961998416066E-15,1.));
#135837=DIRECTION('center_axis',(1.,-9.83319205199467E-31,1.4081690688991E-16));
#135838=DIRECTION('ref_axis',(-1.4081690688991E-16,-6.82961998416066E-15,
1.));
#135839=DIRECTION('center_axis',(-1.,0.,0.));
#135840=DIRECTION('ref_axis',(0.,6.82961998416066E-15,-1.));
#135841=DIRECTION('center_axis',(0.52992421326579,-5.92186660939942E-15,
0.848045003637563));
#135842=DIRECTION('ref_axis',(-0.848045003637563,-3.84166124109038E-15,
0.52992421326579));
#135843=DIRECTION('center_axis',(-0.500005158533422,6.04740227518918E-15,
-0.866022425483294));
#135844=DIRECTION('ref_axis',(0.866022425483294,3.41480999208032E-15,-0.500005158533422));
#135845=DIRECTION('center_axis',(-0.529924185004358,-2.16245522276554E-8,
-0.848045021297494));
#135846=DIRECTION('ref_axis',(-0.848037146343364,-0.00430950302354429,0.529919264233236));
#135847=DIRECTION('center_axis',(0.529924157141051,-5.92186685429947E-15,
0.848045038708645));
#135848=DIRECTION('ref_axis',(-0.848045038708645,-3.84166124109037E-15,
0.529924157141051));
#135849=DIRECTION('center_axis',(-0.500005172385361,-1.05192126270256E-8,
-0.866022417485763));
#135850=DIRECTION('ref_axis',(-0.866013458679397,-0.0045485586909233,0.499999999999984));
#135851=DIRECTION('center_axis',(-0.866037336481536,3.44576744440026E-5,
-0.499979330205396));
#135852=DIRECTION('ref_axis',(0.499979069431911,-0.000963977572674011,-0.866036951219311));
#135853=DIRECTION('center_axis',(1.,-9.83319205199467E-31,1.4081690688991E-16));
#135854=DIRECTION('ref_axis',(-1.4081690688991E-16,-6.82961998416066E-15,
1.));
#135855=DIRECTION('center_axis',(-1.,0.,0.));
#135856=DIRECTION('ref_axis',(0.,6.82961998416066E-15,-1.));
#135857=DIRECTION('center_axis',(-0.529924676825566,-5.22564495945508E-14,
0.848044713969328));
#135858=DIRECTION('ref_axis',(-0.848044713969328,3.84166124109042E-15,-0.529924676825566));
#135859=DIRECTION('center_axis',(-0.529924157141051,5.92186685429947E-15,
-0.848045038708645));
#135860=DIRECTION('ref_axis',(0.848045038708645,3.84166124109037E-15,-0.529924157141051));
#135861=DIRECTION('center_axis',(-0.529924709439995,2.52122320211198E-8,
0.84804469358928));
#135862=DIRECTION('ref_axis',(0.848035979777046,0.00453325469327678,0.529919264233214));
#135863=DIRECTION('center_axis',(-0.529924742154432,6.93661953488301E-14,
0.848044673146739));
#135864=DIRECTION('ref_axis',(-0.848044673146739,3.84166124109097E-15,-0.529924742154432));
#135865=DIRECTION('center_axis',(0.529924185162667,2.16905868611698E-8,
0.84804502119857));
#135866=DIRECTION('ref_axis',(-0.848037146343358,0.0043095030224303,0.529919264233254));
#135867=DIRECTION('center_axis',(-0.52992421326579,5.92186660939942E-15,
-0.848045003637563));
#135868=DIRECTION('ref_axis',(0.848045003637563,3.84166124109038E-15,-0.52992421326579));
#135869=DIRECTION('center_axis',(-1.,0.,0.));
#135870=DIRECTION('ref_axis',(0.,6.82961998416066E-15,-1.));
#135871=DIRECTION('center_axis',(-1.,9.83319205199467E-31,-1.4081690688991E-16));
#135872=DIRECTION('ref_axis',(1.4081690688991E-16,6.82961998416066E-15,
-1.));
#135873=DIRECTION('center_axis',(-0.866018223014801,-3.00422156492971E-5,
0.500012436349089));
#135874=DIRECTION('ref_axis',(0.500012217440556,-0.000989701341688796,0.86601778440251));
#135875=DIRECTION('center_axis',(0.529924742154432,5.92186430159433E-15,
-0.848044673146739));
#135876=DIRECTION('ref_axis',(0.848044673146739,-3.84166124109037E-15,0.529924742154432));
#135877=DIRECTION('center_axis',(0.50000500959944,-1.01138193904953E-8,
-0.866022511471534));
#135878=DIRECTION('ref_axis',(0.866013834616146,-0.00447641077665303,0.499999999999997));
#135879=DIRECTION('center_axis',(-0.50000502301429,-6.04740282155761E-15,
0.866022503726363));
#135880=DIRECTION('ref_axis',(-0.866022503726363,3.41480999208032E-15,-0.50000502301429));
#135881=DIRECTION('center_axis',(0.529924709245831,-2.52894451112192E-8,
-0.848044693710609));
#135882=DIRECTION('ref_axis',(0.848035979777058,-0.0045332546927221,0.5299192642332));
#135883=DIRECTION('center_axis',(0.529924676825566,3.4875337890239E-14,
-0.848044713969328));
#135884=DIRECTION('ref_axis',(0.848044713969328,-3.84166124109041E-15,0.529924676825566));
#135885=DIRECTION('center_axis',(-1.,0.,0.));
#135886=DIRECTION('ref_axis',(0.,6.82961998416066E-15,-1.));
#135887=DIRECTION('center_axis',(1.,0.,0.));
#135888=DIRECTION('ref_axis',(0.,-6.82961998416066E-15,1.));
#135889=DIRECTION('center_axis',(-1.,9.83319205199467E-31,-1.4081690688991E-16));
#135890=DIRECTION('ref_axis',(1.4081690688991E-16,6.82961998416066E-15,
-1.));
#135891=DIRECTION('center_axis',(-1.,-3.81527851617387E-28,5.46369598732844E-14));
#135892=DIRECTION('ref_axis',(-5.46369598732844E-14,6.82961998416066E-15,
-1.));
#135893=DIRECTION('center_axis',(-1.,9.83319205199467E-31,-1.4081690688991E-16));
#135894=DIRECTION('ref_axis',(1.4081690688991E-16,6.82961998416066E-15,
-1.));
#135895=DIRECTION('center_axis',(0.866037336481549,3.44576743629553E-5,
0.499979330205372));
#135896=DIRECTION('ref_axis',(0.499979069431883,0.000963977580906077,-0.866036951219318));
#135897=DIRECTION('center_axis',(-0.500005158533445,6.04740227518909E-15,
-0.866022425483281));
#135898=DIRECTION('ref_axis',(0.86602242548328,3.41480999208034E-15,-0.500005158533445));
#135899=DIRECTION('center_axis',(-0.500005167502186,6.23740986055901E-15,
-0.866022420305105));
#135900=DIRECTION('ref_axis',(5.80463060319271E-12,-1.,-3.35252384988615E-12));
#135901=DIRECTION('center_axis',(0.497265934575139,0.0522647557772062,-0.866022508722875));
#135902=DIRECTION('ref_axis',(-0.104528463271195,0.994521895367901,-2.02375299837496E-12));
#135903=DIRECTION('center_axis',(0.861277224842077,0.0904936763703871,-0.500012436350639));
#135904=DIRECTION('ref_axis',(0.497169646238188,0.0532497883517295,0.86601778440162));
#135905=DIRECTION('center_axis',(-0.497265943181921,-0.0522647566818225,
0.866022503726309));
#135906=DIRECTION('ref_axis',(-0.867207748104376,6.05825588881007E-15,-0.49794650478514));
#135907=DIRECTION('center_axis',(-0.99452189536827,-0.104528463267684,-7.29918357754136E-16));
#135908=DIRECTION('ref_axis',(-0.104528463267684,0.99452189536827,6.82961998416065E-15));
#135909=DIRECTION('center_axis',(0.994521895368273,0.104528463267661,8.69963854894025E-16));
#135910=DIRECTION('ref_axis',(0.104528463267661,-0.994521895368273,-6.82961998416065E-15));
#135911=DIRECTION('center_axis',(0.99452189536827,0.104528463267683,1.60286761075321E-17));
#135912=DIRECTION('ref_axis',(0.104528463267683,-0.99452189536827,-6.82961998416065E-15));
#135913=DIRECTION('center_axis',(0.994521895368273,0.104528463267661,8.69963854894025E-16));
#135914=DIRECTION('ref_axis',(0.104528463267661,-0.994521895368273,-6.82961998416065E-15));
#135915=DIRECTION('center_axis',(-0.99452189536827,-0.104528463267684,-7.29918357754136E-16));
#135916=DIRECTION('ref_axis',(-0.104528463267684,0.99452189536827,6.82961998416065E-15));
#135917=DIRECTION('center_axis',(0.527021232978633,0.0553921636610031,0.848045003637563));
#135918=DIRECTION('ref_axis',(-0.849349030019364,-7.40393733324392E-15,
0.52783162580994));
#135919=DIRECTION('center_axis',(-0.497266077958558,-0.0522647708474047,
-0.866022425483302));
#135920=DIRECTION('ref_axis',(0.86720767039809,7.13435718091396E-15,-0.497946640115905));
#135921=DIRECTION('center_axis',(-0.527021202610616,-0.0553921822221918,
-0.848045021297528));
#135922=DIRECTION('ref_axis',(-0.842941044392581,-0.0929299148441298,0.529919264233154));
#135923=DIRECTION('center_axis',(0.527021177161334,0.0553921577943685,0.848045038708656));
#135924=DIRECTION('ref_axis',(-0.849349064867527,-7.44584183003648E-15,
0.527831569734757));
#135925=DIRECTION('center_axis',(-0.49726609063569,-0.0522647827511846,
-0.866022417485754));
#135926=DIRECTION('ref_axis',(-0.860793892491192,-0.095046697206364,0.500000000000024));
#135927=DIRECTION('center_axis',(-0.861296695145142,-0.0904912830030917,
-0.499979330205271));
#135928=DIRECTION('ref_axis',(0.497340894869072,0.051303347000484,-0.866036951219391));
#135929=DIRECTION('center_axis',(0.104769627595185,-0.994496518411988,-1.37365653674844E-14));
#135930=DIRECTION('ref_axis',(-0.994496518411988,-0.104769627595185,-2.12885829743461E-29));
#135931=DIRECTION('center_axis',(0.994521895368273,0.104528463267661,8.69963854894025E-16));
#135932=DIRECTION('ref_axis',(0.104528463267661,-0.994521895368273,-6.82961998416065E-15));
#135933=DIRECTION('center_axis',(-0.99452189536827,-0.104528463267682,-7.29918357754126E-16));
#135934=DIRECTION('ref_axis',(-0.104528463267682,0.99452189536827,6.82961998416065E-15));
#135935=DIRECTION('center_axis',(-2.80862404029962E-16,-6.99768205256557E-15,
1.));
#135936=DIRECTION('ref_axis',(-1.,2.00430111041611E-30,-2.82080304187759E-16));
#135937=DIRECTION('center_axis',(0.104287292793436,-0.994547213842468,-6.94488607545882E-15));
#135938=DIRECTION('ref_axis',(-0.994547213842468,-0.104287292793436,-3.36172022659011E-29));
#135939=DIRECTION('center_axis',(-0.527021693998993,-0.0553922121162073,
0.84804471396932));
#135940=DIRECTION('ref_axis',(-0.849348742192405,6.20133477398574E-15,-0.527832088960287));
#135941=DIRECTION('center_axis',(-0.527021177161343,-0.0553921577943695,
-0.84804503870865));
#135942=DIRECTION('ref_axis',(0.849349064867521,7.1754696837161E-15,-0.527831569734766));
#135943=DIRECTION('center_axis',(-0.527021729070144,-0.055392190451128,
0.848044693589284));
#135944=DIRECTION('ref_axis',(0.842916495800427,0.0931523188229197,0.529919264233187));
#135945=DIRECTION('center_axis',(-0.527021758969984,-0.0553922189448874,
0.848044673146731));
#135946=DIRECTION('ref_axis',(-0.849348701629304,6.81770145149935E-15,-0.527832154231453));
#135947=DIRECTION('center_axis',(0.527021202762368,0.0553921822932962,0.848045021198576));
#135948=DIRECTION('ref_axis',(-0.843841975853092,-0.0843581245812077,0.529919264233233));
#135949=DIRECTION('center_axis',(-0.527021232978546,-0.0553921636609939,
-0.848045003637618));
#135950=DIRECTION('ref_axis',(0.849349030019419,7.36199811433283E-15,-0.527831625809853));
#135951=DIRECTION('center_axis',(0.104785225574091,-0.994494875050338,-8.01139650341116E-15));
#135952=DIRECTION('ref_axis',(-0.994494875050338,-0.104785225574091,1.5603430202424E-30));
#135953=DIRECTION('center_axis',(-0.99452189536827,-0.104528463267683,-7.29918357754131E-16));
#135954=DIRECTION('ref_axis',(-0.104528463267683,0.99452189536827,6.82961998416065E-15));
#135955=DIRECTION('center_axis',(-2.80862404029962E-16,-6.99768205256557E-15,
1.));
#135956=DIRECTION('ref_axis',(-1.,2.13365834995709E-30,-2.77764288392734E-16));
#135957=DIRECTION('center_axis',(0.104271693993677,-0.994548849394382,-8.04019983285269E-15));
#135958=DIRECTION('ref_axis',(-0.994548849394382,-0.104271693993677,1.6725368118524E-29));
#135959=DIRECTION('center_axis',(-0.994521895368273,-0.104528463267661,
-8.69963854894025E-16));
#135960=DIRECTION('ref_axis',(-0.104528463267661,0.994521895368273,6.82961998416067E-15));
#135961=DIRECTION('center_axis',(-0.861270944309899,-0.0905534316539422,
0.500012436348568));
#135962=DIRECTION('ref_axis',(0.497376550152552,0.0512812290837431,0.866017784402841));
#135963=DIRECTION('center_axis',(0.527021758969972,0.0553922189449323,-0.848044673146736));
#135964=DIRECTION('ref_axis',(0.84934870162931,-6.74368895948955E-15,0.527832154231442));
#135965=DIRECTION('center_axis',(0.497265930897847,0.0522647452191274,-0.866022511471542));
#135966=DIRECTION('ref_axis',(0.861737632557095,0.0860712067703171,0.499999999999995));
#135967=DIRECTION('center_axis',(-0.497265943181812,-0.0522647566818107,
0.866022503726372));
#135968=DIRECTION('ref_axis',(-0.867207748104439,7.38830921412877E-15,-0.497946504785031));
#135969=DIRECTION('center_axis',(0.527021728884924,0.0553921903559162,-0.848044693710608));
#135970=DIRECTION('ref_axis',(0.843864204093765,0.0841354767247419,0.529919264233238));
#135971=DIRECTION('center_axis',(0.527021693998975,0.0553922121162348,-0.848044713969329));
#135972=DIRECTION('ref_axis',(0.849348742192415,-7.50888177194347E-15,0.52783208896027));
#135973=DIRECTION('center_axis',(-0.99452189536827,-0.104528463267683,-1.60286761075321E-17));
#135974=DIRECTION('ref_axis',(-0.104528463267683,0.99452189536827,6.82961998416065E-15));
#135975=DIRECTION('center_axis',(0.99452189536827,0.104528463267683,7.29918357754131E-16));
#135976=DIRECTION('ref_axis',(0.104528463267683,-0.99452189536827,-6.82961998416065E-15));
#135977=DIRECTION('center_axis',(-0.994521895368273,-0.104528463267661,
-8.69963854894025E-16));
#135978=DIRECTION('ref_axis',(-0.104528463267661,0.994521895368273,6.82961998416067E-15));
#135979=DIRECTION('center_axis',(-0.99452189536827,-0.104528463267683,-7.29918357754131E-16));
#135980=DIRECTION('ref_axis',(-0.104528463267683,0.99452189536827,6.82961998416065E-15));
#135981=DIRECTION('center_axis',(-0.994521895368273,-0.104528463267661,
-8.69963854894025E-16));
#135982=DIRECTION('ref_axis',(-0.104528463267661,0.994521895368273,6.82961998416067E-15));
#135983=DIRECTION('center_axis',(0.861289491529725,0.0905598208272782,0.499979330204959));
#135984=DIRECTION('ref_axis',(0.497139368680338,0.0532207406041062,-0.866036951219557));
#135985=DIRECTION('center_axis',(-0.497266077958593,-0.0522647708474091,
-0.866022425483282));
#135986=DIRECTION('ref_axis',(0.86720767039807,6.57816839557369E-15,-0.49794664011594));
#135987=DIRECTION('center_axis',(-0.497266086885392,-0.0522647717856406,
-0.866022420300932));
#135988=DIRECTION('ref_axis',(0.104528463264192,-0.994521895368637,2.01938203211187E-12));
#135989=DIRECTION('center_axis',(0.489078705150196,0.103956887952764,-0.866022508723523));
#135990=DIRECTION('ref_axis',(-0.207911690817648,0.978147600733829,7.86772223991619E-14));
#135991=DIRECTION('center_axis',(0.847099893162016,0.180025927305019,-0.500012436348206));
#135992=DIRECTION('ref_axis',(0.488879980349761,0.104926459536577,0.866017784403032));
#135993=DIRECTION('center_axis',(-0.489078713616374,-0.103956889752297,
0.866022503726307));
#135994=DIRECTION('ref_axis',(-0.8707403454847,2.32007185439358E-16,-0.491743073916842));
#135995=DIRECTION('center_axis',(-0.978147600733806,-0.207911690817757,
-1.45183957723504E-15));
#135996=DIRECTION('ref_axis',(-0.207911690817757,0.978147600733806,6.8296199841607E-15));
#135997=DIRECTION('center_axis',(0.978147600733804,0.207911690817766,1.58957929685223E-15));
#135998=DIRECTION('ref_axis',(0.207911690817766,-0.978147600733804,-6.82961998416066E-15));
#135999=DIRECTION('center_axis',(0.978147600733806,0.207911690817757,-1.38807609986408E-15));
#136000=DIRECTION('ref_axis',(0.207911690817757,-0.978147600733806,-6.8296199841607E-15));
#136001=DIRECTION('center_axis',(0.978147600733804,0.207911690817766,1.58957929685223E-15));
#136002=DIRECTION('ref_axis',(0.207911690817766,-0.978147600733804,-6.82961998416066E-15));
#136003=DIRECTION('center_axis',(-0.978147600733806,-0.207911690817757,
-1.45183957723504E-15));
#136004=DIRECTION('ref_axis',(-0.207911690817757,0.978147600733806,6.8296199841607E-15));
#136005=DIRECTION('center_axis',(0.518344097776651,0.110177439185348,0.848045003637583));
#136006=DIRECTION('ref_axis',(-0.85323958281187,1.15837605560063E-15,0.521519140898037));
#136007=DIRECTION('center_axis',(-0.489078846174,-0.103956917928278,-0.866022425483291));
#136008=DIRECTION('ref_axis',(0.870740269393777,1.51570610952153E-16,-0.4917432086527));
#136009=DIRECTION('center_axis',(-0.518344065636424,-0.11017745446327,-0.848045021297511));
#136010=DIRECTION('ref_axis',(-0.828609503963262,-0.180532167040568,0.52991926423314));
#136011=DIRECTION('center_axis',(0.518344042878403,0.110177427516365,0.848045038708646));
#136012=DIRECTION('ref_axis',(-0.8532396169873,5.9869712929813E-16,0.521519084984783));
#136013=DIRECTION('center_axis',(-0.489078857536072,-0.103956931097839,
-0.866022417485789));
#136014=DIRECTION('ref_axis',(-0.846143288283865,-0.184503484227827,0.499999999999961));
#136015=DIRECTION('center_axis',(-0.847119506978912,-0.180025582247147,
-0.499979330205139));
#136016=DIRECTION('ref_axis',(0.489253749388305,0.1030085813512,-0.866036951219461));
#136017=DIRECTION('center_axis',(0.208148881407623,-0.978097154258592,6.53004781901118E-15));
#136018=DIRECTION('ref_axis',(-0.978097154258592,-0.208148881407623,-2.96788381662184E-29));
#136019=DIRECTION('center_axis',(0.978147600733804,0.207911690817766,1.58957929685223E-15));
#136020=DIRECTION('ref_axis',(0.207911690817766,-0.978147600733804,-6.82961998416066E-15));
#136021=DIRECTION('center_axis',(-0.978147600733806,-0.20791169081776,-1.45183957723506E-15));
#136022=DIRECTION('ref_axis',(-0.20791169081776,0.978147600733805,6.82961998416069E-15));
#136023=DIRECTION('center_axis',(-2.78556626507032E-16,-7.01224015889348E-15,
1.));
#136024=DIRECTION('ref_axis',(-1.,2.00430111041611E-30,-2.75028296583065E-16));
#136025=DIRECTION('center_axis',(0.20767448800183,-0.978197989689806,-6.83072005339165E-15));
#136026=DIRECTION('ref_axis',(-0.978197989689806,-0.20767448800183,3.9702683762468E-29));
#136027=DIRECTION('center_axis',(-0.518344551206579,-0.110177535564846,
0.848044713969321));
#136028=DIRECTION('ref_axis',(-0.853239300541043,-1.24733491466344E-15,
-0.521519602711376));
#136029=DIRECTION('center_axis',(-0.518344042878406,-0.110177427516365,
-0.848045038708644));
#136030=DIRECTION('ref_axis',(0.853239616987299,-6.36492759772716E-16,-0.521519084984785));
#136031=DIRECTION('center_axis',(-0.518344588350029,-0.110177517685333,
0.848044693589281));
#136032=DIRECTION('ref_axis',(0.828561842307981,0.180750786625398,0.529919264233245));
#136033=DIRECTION('center_axis',(-0.518344615107843,-0.110177549147448,
0.848044673146742));
#136034=DIRECTION('ref_axis',(-0.853239260760972,1.43910732930017E-15,-0.521519667794102));
#136035=DIRECTION('center_axis',(0.518344065778186,0.110177454557846,0.848045021198576));
#136036=DIRECTION('ref_axis',(-0.830401496090018,-0.172101506925331,0.529919264233233));
#136037=DIRECTION('center_axis',(-0.518344097776628,-0.110177439185343,
-0.848045003637598));
#136038=DIRECTION('ref_axis',(0.853239582811884,-4.04112561920183E-16,-0.521519140898014));
#136039=DIRECTION('center_axis',(0.208164222161113,-0.978093889466681,4.54346712785195E-15));
#136040=DIRECTION('ref_axis',(-0.978093889466681,-0.208164222161113,4.44186922891595E-30));
#136041=DIRECTION('center_axis',(-0.978147600733806,-0.207911690817757,
4.22799177696351E-15));
#136042=DIRECTION('ref_axis',(-0.207911690817757,0.978147600733806,6.8296199841607E-15));
#136043=DIRECTION('center_axis',(-2.78556626507032E-16,-7.01224015889348E-15,
1.));
#136044=DIRECTION('ref_axis',(-1.,2.13365834995709E-30,-2.77764288392734E-16));
#136045=DIRECTION('center_axis',(0.207659145615657,-0.978201246800563,-8.8463639587112E-15));
#136046=DIRECTION('ref_axis',(-0.978201246800563,-0.207659145615657,3.74304734203989E-29));
#136047=DIRECTION('center_axis',(-0.978147600733804,-0.207911690817766,
-1.58957929685223E-15));
#136048=DIRECTION('ref_axis',(-0.207911690817766,0.978147600733804,6.82961998416068E-15));
#136049=DIRECTION('center_axis',(-0.847087400905467,-0.180084698747548,
0.500012436349562));
#136050=DIRECTION('ref_axis',(0.489291521297893,0.102990311607302,0.866017784402274));
#136051=DIRECTION('center_axis',(0.518344615107832,0.110177549147525,-0.848044673146738));
#136052=DIRECTION('ref_axis',(0.853239260760976,-1.2546710781479E-15,0.521519667794095));
#136053=DIRECTION('center_axis',(0.489078702597484,0.103956877069823,-0.866022511471527));
#136054=DIRECTION('ref_axis',(0.848020052664497,0.175675810170021,0.50000000000001));
#136055=DIRECTION('center_axis',(-0.489078713616299,-0.103956889752283,
0.866022503726351));
#136056=DIRECTION('ref_axis',(-0.870740345484743,8.1185976130115E-16,-0.491743073916766));
#136057=DIRECTION('center_axis',(0.51834458817718,0.110177517564643,-0.84804469371061));
#136058=DIRECTION('ref_axis',(0.830446875605853,0.171882402214531,0.529919264233184));
#136059=DIRECTION('center_axis',(0.518344551206566,0.110177535564845,-0.848044713969329));
#136060=DIRECTION('ref_axis',(0.853239300541051,-1.48217857625388E-15,0.521519602711362));
#136061=DIRECTION('center_axis',(-0.978147600733806,-0.207911690817757,
1.38807609986424E-15));
#136062=DIRECTION('ref_axis',(-0.207911690817757,0.978147600733806,6.8296199841607E-15));
#136063=DIRECTION('center_axis',(0.978147600733807,0.207911690817751,1.45183957723501E-15));
#136064=DIRECTION('ref_axis',(0.207911690817751,-0.978147600733807,-6.82961998416071E-15));
#136065=DIRECTION('center_axis',(-0.978147600733804,-0.207911690817766,
-1.58957929685223E-15));
#136066=DIRECTION('ref_axis',(-0.207911690817766,0.978147600733804,6.82961998416068E-15));
#136067=DIRECTION('center_axis',(-0.978147600733806,-0.207911690817757,
5.76710029884055E-14));
#136068=DIRECTION('ref_axis',(-0.207911690817757,0.978147600733806,6.8296199841607E-15));
#136069=DIRECTION('center_axis',(-0.978147600733804,-0.207911690817766,
-1.58957929685223E-15));
#136070=DIRECTION('ref_axis',(-0.207911690817766,0.978147600733804,6.82961998416068E-15));
#136071=DIRECTION('center_axis',(0.847105178672063,0.180092991630817,0.499979330205193));
#136072=DIRECTION('ref_axis',(0.488852904975831,0.104894406043608,-0.866036951219433));
#136073=DIRECTION('center_axis',(-0.489078846174022,-0.103956917928285,
-0.866022425483278));
#136074=DIRECTION('ref_axis',(0.870740269393764,-6.42192866208513E-16,-0.491743208652722));
#136075=DIRECTION('center_axis',(-0.489078854951574,-0.103956919794024,
-0.866022420302267));
#136076=DIRECTION('ref_axis',(0.207911690820505,-0.978147600733222,-1.63036687875202E-12));
#136077=DIRECTION('center_axis',(0.475533027088661,0.15451004671042,-0.866022508722169));
#136078=DIRECTION('ref_axis',(-0.309016994375666,0.95105651629492,-3.62789414398747E-13));
#136079=DIRECTION('center_axis',(0.823641557784728,0.26758577650676,-0.500012436346558));
#136080=DIRECTION('ref_axis',(0.475234043104007,0.155453534443493,0.866017784404018));
#136081=DIRECTION('center_axis',(-0.47553303531813,-0.154510049384321,0.866022503726307));
#136082=DIRECTION('ref_axis',(-0.876548788012439,1.44209482510565E-15,-0.481313018974061));
#136083=DIRECTION('center_axis',(-0.951056516295146,-0.309016994374972,
-2.15785413849121E-15));
#136084=DIRECTION('ref_axis',(-0.309016994374972,0.951056516295146,6.82961998416073E-15));
#136085=DIRECTION('center_axis',(0.951056516295151,0.309016994374955,2.29177897539327E-15));
#136086=DIRECTION('ref_axis',(0.309016994374955,-0.951056516295151,-6.82961998416066E-15));
#136087=DIRECTION('center_axis',(0.951056516295148,0.309016994374964,2.15785413849116E-15));
#136088=DIRECTION('ref_axis',(0.309016994374964,-0.951056516295148,-6.82961998416075E-15));
#136089=DIRECTION('center_axis',(0.951056516295151,0.309016994374955,2.29177897539327E-15));
#136090=DIRECTION('ref_axis',(0.309016994374955,-0.951056516295151,-6.82961998416066E-15));
#136091=DIRECTION('center_axis',(-0.951056516295151,-0.309016994374956,
-2.1578541384911E-15));
#136092=DIRECTION('ref_axis',(-0.309016994374956,0.951056516295151,6.82961998416057E-15));
#136093=DIRECTION('center_axis',(0.503987876168974,0.163755587629894,0.848045003637587));
#136094=DIRECTION('ref_axis',(-0.859649462041495,-7.24230631194929E-16,
0.510884333691853));
#136095=DIRECTION('center_axis',(-0.475533164204393,-0.154510091261976,
-0.866022425483297));
#136096=DIRECTION('ref_axis',(0.876548714628846,1.87535286613278E-16,-0.481313152617418));
#136097=DIRECTION('center_axis',(-0.503987842609475,-0.163755599459623,
-0.848045021297494));
#136098=DIRECTION('ref_axis',(-0.805199544417973,-0.266156471015856,0.529919264233218));
#136099=DIRECTION('center_axis',(0.503987822791202,0.163755570286405,0.848045038708652));
#136100=DIRECTION('ref_axis',(-0.859649495083705,-1.79266124745912E-15,
0.510884278092732));
#136101=DIRECTION('center_axis',(-0.475533174129345,-0.154510105541947,
-0.866022417485764));
#136102=DIRECTION('ref_axis',(-0.822222161144011,-0.271938812462805,0.499999999999991));
#136103=DIRECTION('center_axis',(-0.8236611002229,-0.267587483539854,-0.49997933020517));
#136104=DIRECTION('ref_axis',(0.475806237445598,0.153585232136407,-0.866036951219444));
#136105=DIRECTION('center_axis',(0.309247612517411,-0.950981553003149,-3.26200391676225E-14));
#136106=DIRECTION('ref_axis',(-0.950981553003149,-0.309247612517411,-3.41480999208011E-15));
#136107=DIRECTION('center_axis',(0.951056516295151,0.309016994374955,2.29177897539327E-15));
#136108=DIRECTION('ref_axis',(0.309016994374955,-0.951056516295151,-6.82961998416066E-15));
#136109=DIRECTION('center_axis',(-0.951056516295151,-0.309016994374956,
-2.1578541384911E-15));
#136110=DIRECTION('ref_axis',(-0.309016994374956,0.951056516295151,6.82961998416057E-15));
#136111=DIRECTION('center_axis',(-2.74741743792087E-16,-7.02647749501057E-15,
1.));
#136112=DIRECTION('ref_axis',(-1.,2.00430111041611E-30,-2.75028296583065E-16));
#136113=DIRECTION('center_axis',(0.308786358060997,-0.951131423661013,-6.64171523299946E-15));
#136114=DIRECTION('ref_axis',(-0.951131423661013,-0.308786358060997,-3.41480999208026E-15));
#136115=DIRECTION('center_axis',(-0.503988317040562,-0.16375573087774,0.848044713969328));
#136116=DIRECTION('ref_axis',(-0.859649189130478,-2.03018390514586E-16,
-0.510884792910606));
#136117=DIRECTION('center_axis',(-0.503987822791237,-0.163755570286416,
-0.848045038708628));
#136118=DIRECTION('ref_axis',(0.859649495083683,4.98171905108308E-17,-0.510884278092769));
#136119=DIRECTION('center_axis',(-0.503988355851731,-0.163755716971875,
0.848044693589256));
#136120=DIRECTION('ref_axis',(0.805129291876083,0.266368911019414,0.529919264233193));
#136121=DIRECTION('center_axis',(-0.503988379172014,-0.163755751065428,
0.848044673146742));
#136122=DIRECTION('ref_axis',(-0.859649150669462,-1.65774526852702E-15,
-0.510884857627698));
#136123=DIRECTION('center_axis',(0.503987842737129,0.163755599579094,0.84804502119856));
#136124=DIRECTION('ref_axis',(-0.807862963764753,-0.25795930913955,0.529919264233219));
#136125=DIRECTION('center_axis',(-0.50398787616897,-0.163755587629893,-0.84804500363759));
#136126=DIRECTION('ref_axis',(0.859649462041497,1.07198038077594E-15,-0.510884333691849));
#136127=DIRECTION('center_axis',(0.309262527968972,-0.95097670255072,-6.64063482126083E-15));
#136128=DIRECTION('ref_axis',(-0.95097670255072,-0.309262527968972,-3.41480999208037E-15));
#136129=DIRECTION('center_axis',(-0.951056516295148,-0.309016994374964,
-2.15785413849116E-15));
#136130=DIRECTION('ref_axis',(-0.309016994374964,0.951056516295148,6.82961998416075E-15));
#136131=DIRECTION('center_axis',(-2.74741743792087E-16,-7.02647749501057E-15,
1.));
#136132=DIRECTION('ref_axis',(-1.,2.13365834995709E-30,-2.77764288392734E-16));
#136133=DIRECTION('center_axis',(0.308771440182806,-0.951136266645025,-6.64174905137606E-15));
#136134=DIRECTION('ref_axis',(-0.951136266645025,-0.308771440182806,-3.41480999208035E-15));
#136135=DIRECTION('center_axis',(-0.951056516295151,-0.309016994374955,
-2.29177897539327E-15));
#136136=DIRECTION('ref_axis',(-0.309016994374955,0.951056516295151,6.82961998416058E-15));
#136137=DIRECTION('center_axis',(-0.823622990672772,-0.267642920195548,
0.500012436349775));
#136138=DIRECTION('ref_axis',(0.475845712151136,0.153571010697317,0.866017784402135));
#136139=DIRECTION('center_axis',(0.503988379171984,0.163755751065574,-0.848044673146731));
#136140=DIRECTION('ref_axis',(0.859649150669472,-1.91145464518171E-15,0.51088485762768));
#136141=DIRECTION('center_axis',(0.475533025685305,0.154510035619257,-0.866022511471564));
#136142=DIRECTION('ref_axis',(0.825011387615606,0.263355672626591,0.499999999999969));
#136143=DIRECTION('center_axis',(-0.475533035318107,-0.154510049384286,
0.866022503726325));
#136144=DIRECTION('ref_axis',(-0.876548788012453,5.44148765414771E-16,-0.481313018974035));
#136145=DIRECTION('center_axis',(0.503988355690328,0.163755716840074,-0.848044693710628));
#136146=DIRECTION('ref_axis',(0.807930997361746,0.257746148170262,0.529919264233192));
#136147=DIRECTION('center_axis',(0.503988317040544,0.163755730877811,-0.848044713969325));
#136148=DIRECTION('ref_axis',(0.859649189130485,7.79100967592155E-16,0.510884792910593));
#136149=DIRECTION('center_axis',(-0.951056516295148,-0.309016994374964,
-2.15785413849116E-15));
#136150=DIRECTION('ref_axis',(-0.309016994374964,0.951056516295148,6.82961998416075E-15));
#136151=DIRECTION('center_axis',(0.951056516295148,0.309016994374964,2.15785413849116E-15));
#136152=DIRECTION('ref_axis',(0.309016994374964,-0.951056516295148,-6.82961998416075E-15));
#136153=DIRECTION('center_axis',(-0.951056516295151,-0.309016994374955,
-2.29177897539327E-15));
#136154=DIRECTION('ref_axis',(-0.309016994374955,0.951056516295151,6.82961998416058E-15));
#136155=DIRECTION('center_axis',(-0.951056516295148,-0.309016994374964,
6.28402042242275E-15));
#136156=DIRECTION('ref_axis',(-0.309016994374964,0.951056516295148,6.82961998416068E-15));
#136157=DIRECTION('center_axis',(-0.951056516295151,-0.309016994374955,
-2.29177897539327E-15));
#136158=DIRECTION('ref_axis',(-0.309016994374955,0.951056516295151,6.82961998416058E-15));
#136159=DIRECTION('center_axis',(0.823639804208761,0.267653025931831,0.499979330205248));
#136160=DIRECTION('ref_axis',(0.475210466541244,0.155418826440911,-0.866036951219394));
#136161=DIRECTION('center_axis',(-0.47553316420442,-0.154510091261976,-0.866022425483283));
#136162=DIRECTION('ref_axis',(0.876548714628831,-9.05295501398111E-16,-0.481313152617445));
#136163=DIRECTION('center_axis',(-0.475533172737204,-0.154510094034435,
-0.866022420303284));
#136164=DIRECTION('ref_axis',(0.309016994382667,-0.951056516292645,-4.69440758122482E-12));
#136165=DIRECTION('center_axis',(0.456777309668931,0.203370361062697,-0.866022508721824));
#136166=DIRECTION('ref_axis',(-0.406736643079858,0.913545457640795,-2.53078398719129E-12));
#136167=DIRECTION('center_axis',(0.791159233140771,0.352213899940676,-0.500012436350025));
#136168=DIRECTION('ref_axis',(0.456381342224756,0.204277427946829,0.866017784402005));
#136169=DIRECTION('center_axis',(-0.456777317573273,-0.203370364581918,
0.866022503726308));
#136170=DIRECTION('ref_axis',(-0.884507036382098,-9.28493662905854E-16,
-0.466526850878444));
#136171=DIRECTION('center_axis',(-0.913545457642594,-0.406736643075817,
-2.84022679824583E-15));
#136172=DIRECTION('ref_axis',(-0.406736643075817,0.913545457642593,6.82961998416057E-15));
#136173=DIRECTION('center_axis',(0.913545457642598,0.406736643075807,2.96886944389432E-15));
#136174=DIRECTION('ref_axis',(0.406736643075807,-0.913545457642598,-6.82961998416066E-15));
#136175=DIRECTION('center_axis',(0.913545457642598,0.406736643075807,2.84022679824576E-15));
#136176=DIRECTION('ref_axis',(0.406736643075807,-0.913545457642598,-6.8296199841606E-15));
#136177=DIRECTION('center_axis',(0.913545457642598,0.406736643075807,2.96886944389432E-15));
#136178=DIRECTION('ref_axis',(0.406736643075807,-0.913545457642598,-6.82961998416066E-15));
#136179=DIRECTION('center_axis',(-0.913545457642594,-0.406736643075817,
-2.84022679824583E-15));
#136180=DIRECTION('ref_axis',(-0.406736643075817,0.913545457642593,6.82961998416057E-15));
#136181=DIRECTION('center_axis',(0.484109857923749,0.215539595588291,0.848045003637592));
#136182=DIRECTION('ref_axis',(-0.868458021516008,-1.07236589050538E-15,
0.495762710239991));
#136183=DIRECTION('center_axis',(-0.456777441376078,-0.203370419702497,
-0.866022425483286));
#136184=DIRECTION('ref_axis',(0.884506966812055,-2.08482502526669E-15,-0.466526982779066));
#136185=DIRECTION('center_axis',(-0.484109823308942,-0.215539603851087,
-0.848045021297514));
#136186=DIRECTION('ref_axis',(-0.77296765015055,-0.348864709042549,0.529919264233142));
#136187=DIRECTION('center_axis',(0.484109806651292,0.215539572760322,0.848045038708645));
#136188=DIRECTION('ref_axis',(-0.868458052949955,-5.26259601010897E-16,
0.495762655175208));
#136189=DIRECTION('center_axis',(-0.456777449753612,-0.203370434942479,
-0.866022417485768));
#136190=DIRECTION('ref_axis',(-0.789292595944142,-0.356394722166,0.499999999999978));
#136191=DIRECTION('center_axis',(-0.791178490090692,-0.352217640366598,
-0.499979330205158));
#136192=DIRECTION('ref_axis',(0.457145692798374,0.20247917097425,-0.866036951219447));
#136193=DIRECTION('center_axis',(0.406958162070226,-0.913446798847324,-6.37856490440286E-15));
#136194=DIRECTION('ref_axis',(-0.913446798847324,-0.406958162070226,-3.41480999208029E-15));
#136195=DIRECTION('center_axis',(0.913545457642598,0.406736643075807,2.96886944389432E-15));
#136196=DIRECTION('ref_axis',(0.406736643075807,-0.913545457642598,-6.82961998416066E-15));
#136197=DIRECTION('center_axis',(-0.913545457642603,-0.406736643075797,
-2.84022679824569E-15));
#136198=DIRECTION('ref_axis',(-0.406736643075797,0.913545457642603,6.82961998416064E-15));
#136199=DIRECTION('center_axis',(-2.69459552538469E-16,-7.04023807368299E-15,
1.));
#136200=DIRECTION('ref_axis',(-1.,2.00430111041611E-30,-2.67976288978371E-16));
#136201=DIRECTION('center_axis',(0.406515100163544,-0.913644062717546,-6.37994239064628E-15));
#136202=DIRECTION('ref_axis',(-0.913644062717546,-0.406515100163544,-3.41480999208035E-15));
#136203=DIRECTION('center_axis',(-0.484110281406756,-0.215539784135086,
0.8480447139693));
#136204=DIRECTION('ref_axis',(-0.868457761888263,3.97238567950502E-16,-0.495763165045598));
#136205=DIRECTION('center_axis',(-0.48410980665131,-0.215539572760331,-0.848045038708632));
#136206=DIRECTION('ref_axis',(0.868458052949944,-6.20882257334192E-16,-0.495762655175228));
#136207=DIRECTION('center_axis',(-0.484110321456857,-0.215539774366594,
0.84804469358928));
#136208=DIRECTION('ref_axis',(0.772875576437733,0.349068641875244,0.529919264233161));
#136209=DIRECTION('center_axis',(-0.484110341087621,-0.215539810706668,
0.84804467314674));
#136210=DIRECTION('ref_axis',(-0.868457725299266,-4.18857327554064E-16,
-0.495763229140711));
#136211=DIRECTION('center_axis',(0.484109823426014,0.215539603977446,0.848045021198568));
#136212=DIRECTION('ref_axis',(-0.776473315749786,-0.340990855189784,0.529919264233215));
#136213=DIRECTION('center_axis',(-0.484109857923765,-0.215539595588298,
-0.848045003637581));
#136214=DIRECTION('ref_axis',(0.868458021515998,4.63801329176873E-17,-0.495762710240007));
#136215=DIRECTION('center_axis',(0.406972488803041,-0.913440415876952,-6.37852033235898E-15));
#136216=DIRECTION('ref_axis',(-0.913440415876952,-0.406972488803041,-3.41480999208023E-15));
#136217=DIRECTION('center_axis',(-0.913545457642598,-0.406736643075807,
-2.84022679824576E-15));
#136218=DIRECTION('ref_axis',(-0.406736643075807,0.913545457642598,6.82961998416061E-15));
#136219=DIRECTION('center_axis',(-2.69459552538469E-16,-7.04023807368299E-15,
1.));
#136220=DIRECTION('ref_axis',(-1.,2.13365834995709E-30,-2.70257145463201E-16));
#136221=DIRECTION('center_axis',(0.40650077023674,-0.913650438514062,-6.37998691259538E-15));
#136222=DIRECTION('ref_axis',(-0.913650438514062,-0.40650077023674,-3.41480999208026E-15));
#136223=DIRECTION('center_axis',(-0.913545457642598,-0.406736643075807,
-2.96886944389432E-15));
#136224=DIRECTION('ref_axis',(-0.406736643075807,0.913545457642598,6.8296199841606E-15));
#136225=DIRECTION('center_axis',(-0.791134794600364,-0.352268789801749,
0.500012436349588));
#136226=DIRECTION('ref_axis',(0.457186437802727,0.202469153671098,0.866017784402238));
#136227=DIRECTION('center_axis',(0.484110341087585,0.21553981070676,-0.848044673146738));
#136228=DIRECTION('ref_axis',(0.868457725299281,1.87917867469974E-15,0.495763229140685));
#136229=DIRECTION('center_axis',(0.456777309429339,0.203370349891571,-0.86602251147154));
#136230=DIRECTION('ref_axis',(0.792963725156868,0.34815015522809,0.499999999999999));
#136231=DIRECTION('center_axis',(-0.456777317573209,-0.203370364581889,
0.866022503726348));
#136232=DIRECTION('ref_axis',(-0.884507036382134,8.46452346853348E-16,-0.466526850878376));
#136233=DIRECTION('center_axis',(0.484110321308894,0.215539774221645,-0.848044693710586));
#136234=DIRECTION('ref_axis',(0.776563258034758,0.340785973398144,0.529919264233261));
#136235=DIRECTION('center_axis',(0.4841102814067,0.215539784135111,-0.848044713969326));
#136236=DIRECTION('ref_axis',(0.868457761888295,-2.69120973473327E-15,0.495763165045542));
#136237=DIRECTION('center_axis',(-0.913545457642598,-0.406736643075807,
-2.84022679824576E-15));
#136238=DIRECTION('ref_axis',(-0.406736643075807,0.913545457642598,6.82961998416061E-15));
#136239=DIRECTION('center_axis',(0.913545457642598,0.406736643075807,2.84022679824576E-15));
#136240=DIRECTION('ref_axis',(0.406736643075807,-0.913545457642598,-6.8296199841606E-15));
#136241=DIRECTION('center_axis',(-0.913545457642598,-0.406736643075807,
-2.96886944389432E-15));
#136242=DIRECTION('ref_axis',(-0.406736643075807,0.913545457642598,6.8296199841606E-15));
#136243=DIRECTION('center_axis',(-0.913545457642598,-0.406736643075807,
4.70731197133941E-14));
#136244=DIRECTION('ref_axis',(-0.406736643075807,0.913545457642598,6.82961998416061E-15));
#136245=DIRECTION('center_axis',(-0.913545457642598,-0.406736643075807,
-2.96886944389432E-15));
#136246=DIRECTION('ref_axis',(-0.406736643075807,0.913545457642598,6.8296199841606E-15));
#136247=DIRECTION('center_axis',(0.791150459692853,0.352280597671104,0.499979330205037));
#136248=DIRECTION('ref_axis',(0.456361522798632,0.204240445630384,-0.866036951219528));
#136249=DIRECTION('center_axis',(-0.456777441376069,-0.203370419702462,
-0.866022425483299));
#136250=DIRECTION('ref_axis',(0.884506966812061,-1.67212674088141E-15,-0.466526982779053));
#136251=DIRECTION('center_axis',(-0.456777449577965,-0.203370423354209,
-0.866022420299717));
#136252=DIRECTION('ref_axis',(0.406736643067868,-0.913545457646133,5.02660029630347E-12));
#136253=DIRECTION('center_axis',(0.43301704445322,0.250002507178805,-0.866022508724404));
#136254=DIRECTION('ref_axis',(-0.499999999998154,0.866025403785504,1.25883555838488E-12));
#136255=DIRECTION('center_axis',(0.750008802379566,0.432983094185441,-0.500012436348108));
#136256=DIRECTION('ref_axis',(0.432528431860175,0.250863215179282,0.866017784403121));
#136257=DIRECTION('center_axis',(-0.433017051950279,-0.250002511507204,
0.866022503726306));
#136258=DIRECTION('ref_axis',(-0.894424794863783,8.12848018235645E-16,-0.447218387740128));
#136259=DIRECTION('center_axis',(-0.86602540378444,-0.499999999999998,-3.49148133884312E-15));
#136260=DIRECTION('ref_axis',(-0.499999999999998,0.86602540378444,6.82961998416073E-15));
#136261=DIRECTION('center_axis',(0.866025403784435,0.500000000000007,3.61343235749219E-15));
#136262=DIRECTION('ref_axis',(0.500000000000007,-0.866025403784434,-6.82961998416066E-15));
#136263=DIRECTION('center_axis',(0.866025403784433,0.50000000000001,1.71507213071646E-14));
#136264=DIRECTION('ref_axis',(0.50000000000001,-0.866025403784433,-6.82961998416028E-15));
#136265=DIRECTION('center_axis',(0.866025403784435,0.500000000000007,3.61343235749219E-15));
#136266=DIRECTION('ref_axis',(0.500000000000007,-0.866025403784434,-6.82961998416066E-15));
#136267=DIRECTION('center_axis',(-0.866025403784433,-0.50000000000001,-3.4914813388432E-15));
#136268=DIRECTION('ref_axis',(-0.50000000000001,0.866025403784433,6.82961998416068E-15));
#136269=DIRECTION('center_axis',(0.458927830768604,0.264962106632857,0.848045003637603));
#136270=DIRECTION('ref_axis',(-0.879478602053345,-2.33963297980692E-15,
0.475938429348056));
#136271=DIRECTION('center_axis',(-0.433017169313214,-0.250002579266714,
-0.866022425483291));
#136272=DIRECTION('ref_axis',(0.894424730216418,1.24757342180764E-15,-0.447218517033103));
#136273=DIRECTION('center_axis',(-0.458927795481002,-0.264962111230046,
-0.848045021297492));
#136274=DIRECTION('ref_axis',(-0.73226696057136,-0.42775071227305,0.529919264233224));
#136275=DIRECTION('center_axis',(0.45892778216323,0.264962078570532,0.84804503870863));
#136276=DIRECTION('ref_axis',(-0.879478631391236,9.86399431822428E-16,0.475938375135058));
#136277=DIRECTION('center_axis',(-0.433017176052355,-0.250002595298109,
-0.866022417485745));
#136278=DIRECTION('ref_axis',(-0.74771537589394,-0.436945896710048,0.500000000000037));
#136279=DIRECTION('center_axis',(-0.750027562856189,-0.432988827019237,
-0.499979330205271));
#136280=DIRECTION('ref_axis',(0.433476564277263,0.249154705644953,-0.866036951219379));
#136281=DIRECTION('center_axis',(0.500209992837911,-0.865904130412309,-6.04657622512354E-15));
#136282=DIRECTION('ref_axis',(-0.865904130412309,-0.500209992837911,-3.41480999208024E-15));
#136283=DIRECTION('center_axis',(0.866025403784435,0.500000000000007,3.61343235749219E-15));
#136284=DIRECTION('ref_axis',(0.500000000000007,-0.866025403784434,-6.82961998416066E-15));
#136285=DIRECTION('center_axis',(-0.86602540378444,-0.499999999999998,-3.49148133884312E-15));
#136286=DIRECTION('ref_axis',(-0.499999999999998,0.86602540378444,6.82961998416073E-15));
#136287=DIRECTION('center_axis',(-2.6276792553892E-16,-7.05337113113122E-15,
1.));
#136288=DIRECTION('ref_axis',(-1.,2.00430111041611E-30,-2.60924281373677E-16));
#136289=DIRECTION('center_axis',(0.499789977759954,-0.866146626230631,-6.04826956437238E-15));
#136290=DIRECTION('ref_axis',(-0.866146626230631,-0.499789977759954,-3.41480999208016E-15));
#136291=DIRECTION('center_axis',(-0.458928232223265,-0.26496233841278,0.848044713969294));
#136292=DIRECTION('ref_axis',(-0.879478359737711,-6.74342126943788E-16,
-0.475938877118759));
#136293=DIRECTION('center_axis',(-0.458927782163224,-0.264962078570537,
-0.848045038708632));
#136294=DIRECTION('ref_axis',(0.879478631391239,-9.21361465146423E-16,-0.475938375135052));
#136295=DIRECTION('center_axis',(-0.45892827307447,-0.264962332885157,0.848044693589283));
#136296=DIRECTION('ref_axis',(0.732154074464099,0.427943903613708,0.529919264233223));
#136297=DIRECTION('center_axis',(-0.458928288799681,-0.264962371077198,
0.848044673146731));
#136298=DIRECTION('ref_axis',(-0.879478325588497,1.93561850010889E-15,-0.475938940222435));
#136299=DIRECTION('center_axis',(0.458927795581622,0.264962111372437,0.848045021198552));
#136300=DIRECTION('ref_axis',(-0.736576463604389,-0.420286434064426,0.529919264233204));
#136301=DIRECTION('center_axis',(-0.458927830768623,-0.264962106632877,
-0.848045003637587));
#136302=DIRECTION('ref_axis',(0.879478602053333,4.74704422624339E-16,-0.475938429348078));
#136303=DIRECTION('center_axis',(0.500223573885336,-0.865896284857131,-2.60257666760256E-14));
#136304=DIRECTION('ref_axis',(-0.865896284857131,-0.500223573885336,-3.41480999208053E-15));
#136305=DIRECTION('center_axis',(-0.866025403784433,-0.50000000000001,-3.4914813388432E-15));
#136306=DIRECTION('ref_axis',(-0.50000000000001,0.866025403784433,6.82961998416068E-15));
#136307=DIRECTION('center_axis',(-2.6276792553892E-16,-7.05337113113122E-15,
1.));
#136308=DIRECTION('ref_axis',(-1.,1.70692667996567E-30,-2.62750002533667E-16));
#136309=DIRECTION('center_axis',(0.499776392786197,-0.866154464985095,-2.40408495755615E-15));
#136310=DIRECTION('ref_axis',(-0.866154464985095,-0.499776392786197,-3.4148099920803E-15));
#136311=DIRECTION('center_axis',(-0.866025403784435,-0.500000000000007,
-3.61343235749219E-15));
#136312=DIRECTION('ref_axis',(-0.500000000000007,0.866025403784435,6.82961998416069E-15));
#136313=DIRECTION('center_axis',(-0.749978760162892,-0.43303512882955,0.500012436349444));
#136314=DIRECTION('ref_axis',(-0.433518133162554,-0.249149002241894,-0.866017784402331));
#136315=DIRECTION('center_axis',(0.458928288799652,0.264962371077227,-0.848044673146738));
#136316=DIRECTION('ref_axis',(0.87947832558851,-9.67081701894375E-18,0.47593894022241));
#136317=DIRECTION('center_axis',(0.433017045388799,0.250002496042169,-0.866022511471521));
#136318=DIRECTION('ref_axis',(0.752228186192834,0.42913023186094,0.500000000000015));
#136319=DIRECTION('center_axis',(-0.433017051950174,-0.250002511507144,
0.866022503726376));
#136320=DIRECTION('ref_axis',(-0.89442479486384,8.04235003406217E-16,-0.447218387740013));
#136321=DIRECTION('center_axis',(0.458928272945295,0.264962332720549,-0.848044693710617));
#136322=DIRECTION('ref_axis',(0.736687329162614,0.420092076152143,0.529919264233182));
#136323=DIRECTION('center_axis',(0.458928232223185,0.264962338412833,-0.84804471396932));
#136324=DIRECTION('ref_axis',(0.879478359737753,-7.9487078306857E-16,0.475938877118682));
#136325=DIRECTION('center_axis',(-0.866025403784433,-0.50000000000001,-3.4914813388432E-15));
#136326=DIRECTION('ref_axis',(-0.50000000000001,0.866025403784433,6.82961998416068E-15));
#136327=DIRECTION('center_axis',(0.866025403784433,0.50000000000001,3.4914813388432E-15));
#136328=DIRECTION('ref_axis',(0.50000000000001,-0.866025403784433,-6.82961998416068E-15));
#136329=DIRECTION('center_axis',(-0.866025403784435,-0.500000000000007,
-3.61343235749219E-15));
#136330=DIRECTION('ref_axis',(-0.500000000000007,0.866025403784435,6.82961998416069E-15));
#136331=DIRECTION('center_axis',(-0.866025403784433,-0.50000000000001,3.74862385661209E-14));
#136332=DIRECTION('ref_axis',(-0.50000000000001,0.866025403784433,6.82961998416068E-15));
#136333=DIRECTION('center_axis',(-0.866025403784435,-0.500000000000007,
-3.61343235749219E-15));
#136334=DIRECTION('ref_axis',(-0.500000000000007,0.866025403784435,6.82961998416069E-15));
#136335=DIRECTION('center_axis',(0.74999310518165,0.433048509462076,0.49997933020542));
#136336=DIRECTION('ref_axis',(-0.432512586705212,-0.25082436377741,0.866036951219302));
#136337=DIRECTION('center_axis',(-0.433017169313192,-0.250002579266702,
-0.866022425483305));
#136338=DIRECTION('ref_axis',(0.89442473021643,2.60762584234072E-15,-0.44721851703308));
#136339=DIRECTION('center_axis',(-0.433017177087641,-0.250002583755266,
-0.866022420300272));
#136340=DIRECTION('ref_axis',(0.500000000001662,-0.866025403783479,-1.11022302198922E-12));
#136341=DIRECTION('center_axis',(0.404512553890246,0.293895573513346,-0.866022508722754));
#136342=DIRECTION('ref_axis',(-0.587785252293392,0.80901699437428,-6.3815969278833E-13));
#136343=DIRECTION('center_axis',(0.7006411182289,0.509008435040742,-0.500012436349669));
#136344=DIRECTION('ref_axis',(0.403936649482838,0.294700492540559,0.866017784402221));
#136345=DIRECTION('center_axis',(-0.404512560891457,-0.293895578600025,
0.866022503726313));
#136346=DIRECTION('ref_axis',(-0.906035256115487,1.67656260149152E-15,-0.423202214875755));
#136347=DIRECTION('center_axis',(-0.80901699437495,-0.58778525229247,2.80103167643593E-14));
#136348=DIRECTION('ref_axis',(-0.58778525229247,0.80901699437495,6.82961998416043E-15));
#136349=DIRECTION('center_axis',(0.809016994374943,0.58778525229248,4.21840575002204E-15));
#136350=DIRECTION('ref_axis',(0.58778525229248,-0.809016994374943,-6.82961998416066E-15));
#136351=DIRECTION('center_axis',(0.809016994374931,0.587785252292496,4.83067115377211E-14));
#136352=DIRECTION('ref_axis',(0.587785252292496,-0.809016994374931,-6.82961998416074E-15));
#136353=DIRECTION('center_axis',(0.809016994374943,0.58778525229248,4.21840575002204E-15));
#136354=DIRECTION('ref_axis',(0.58778525229248,-0.809016994374943,-6.82961998416066E-15));
#136355=DIRECTION('center_axis',(-0.80901699437495,-0.58778525229247,-4.10448247925272E-15));
#136356=DIRECTION('ref_axis',(-0.58778525229247,0.80901699437495,6.82961998416043E-15));
#136357=DIRECTION('center_axis',(0.428717694262752,0.311481637390302,0.848045003637594));
#136358=DIRECTION('ref_axis',(-0.892442058026275,-9.10482188530049E-16,
0.451162025292274));
#136359=DIRECTION('center_axis',(-0.404512670528681,-0.293895658256099,
-0.866022425483295));
#136360=DIRECTION('ref_axis',(0.906035197473496,2.00150227313137E-15,-0.423202340422597));
#136361=DIRECTION('center_axis',(-0.428717658683062,-0.311481638280321,
-0.848045021297526));
#136362=DIRECTION('ref_axis',(-0.683543400924993,-0.501950189208491,0.529919264233199));
#136363=DIRECTION('center_axis',(0.428717648856917,0.311481604401031,0.848045038708651));
#136364=DIRECTION('ref_axis',(-0.892442084777737,-1.93926946889151E-15,
0.451161972375294));
#136365=DIRECTION('center_axis',(-0.404512675554545,-0.293895674904908,
-0.866022417485767));
#136366=DIRECTION('ref_axis',(-0.697946029716633,-0.512709800572198,0.500000000000006));
#136367=DIRECTION('center_axis',(-0.700659176690448,-0.509016097473817,
-0.499979330204749));
#136368=DIRECTION('ref_axis',(0.405058175797697,0.293100449234632,-0.866036951219692));
#136369=DIRECTION('center_axis',(0.587981418248444,-0.808874435122379,-5.64833999139414E-15));
#136370=DIRECTION('ref_axis',(-0.808874435122379,-0.587981418248444,-3.41480999208026E-15));
#136371=DIRECTION('center_axis',(0.809016994374943,0.58778525229248,4.21840575002204E-15));
#136372=DIRECTION('ref_axis',(0.58778525229248,-0.809016994374943,-6.82961998416066E-15));
#136373=DIRECTION('center_axis',(-0.809016994374912,-0.587785252292522,
-4.10448247925309E-15));
#136374=DIRECTION('ref_axis',(-0.587785252292522,0.809016994374912,6.82961998416056E-15));
#136375=DIRECTION('center_axis',(-2.54740177659162E-16,-7.0657327788296E-15,
1.));
#136376=DIRECTION('ref_axis',(-1.,2.00430111041611E-30,-2.53872273768983E-16));
#136377=DIRECTION('center_axis',(0.587589051772227,-0.809159506053914,-5.65033063106954E-15));
#136378=DIRECTION('ref_axis',(-0.809159506053914,-0.587589051772227,-3.41480999208049E-15));
#136379=DIRECTION('center_axis',(-0.428718069290599,-0.311481909863915,
0.848044713969298));
#136380=DIRECTION('ref_axis',(-0.892441837073364,8.23210690846008E-16,-0.451162462358205));
#136381=DIRECTION('center_axis',(-0.428717648856922,-0.311481604401035,
-0.848045038708647));
#136382=DIRECTION('ref_axis',(0.892442084777735,8.95023997870107E-16,-0.4511619723753));
#136383=DIRECTION('center_axis',(-0.428718110495355,-0.31148190863732,0.848044693589286));
#136384=DIRECTION('ref_axis',(0.683410939224747,0.502130522416714,0.529919264233211));
#136385=DIRECTION('center_axis',(-0.428718122142699,-0.311481948263271,
0.848044673146736));
#136386=DIRECTION('ref_axis',(-0.892441805934777,1.08348165947679E-15,-0.451162523953258));
#136387=DIRECTION('center_axis',(0.428717658780688,0.311481638415343,0.848045021198579));
#136388=DIRECTION('ref_axis',(-0.688609525569338,-0.494977266841255,0.529919264233272));
#136389=DIRECTION('center_axis',(-0.428717694262775,-0.311481637390318,
-0.848045003637576));
#136390=DIRECTION('ref_axis',(0.892442058026262,-8.62993040855731E-16,-0.4511620252923));
#136391=DIRECTION('center_axis',(0.587994104813606,-0.808865212939984,-5.64827559323867E-15));
#136392=DIRECTION('ref_axis',(-0.808865212939984,-0.587994104813606,-3.41480999208028E-15));
#136393=DIRECTION('center_axis',(-0.809016994374931,-0.587785252292496,
-4.1044824792529E-15));
#136394=DIRECTION('ref_axis',(-0.587785252292496,0.809016994374931,6.82961998416073E-15));
#136395=DIRECTION('center_axis',(-2.54740177659162E-16,-7.0657327788296E-15,
1.));
#136396=DIRECTION('ref_axis',(-1.,1.70692667996567E-30,-2.55242859604134E-16));
#136397=DIRECTION('center_axis',(0.587576360591375,-0.809168721883263,-1.77575279369932E-14));
#136398=DIRECTION('ref_axis',(-0.809168721883263,-0.587576360591375,-3.41480999208057E-15));
#136399=DIRECTION('center_axis',(-0.809016994374943,-0.58778525229248,-4.21840575002204E-15));
#136400=DIRECTION('ref_axis',(-0.58778525229248,0.809016994374943,6.8296199841606E-15));
#136401=DIRECTION('center_axis',(-0.70060580148539,-0.50905704436808,0.500012436349587));
#136402=DIRECTION('ref_axis',(-0.40510011312848,-0.29309912221343,-0.866017784402266));
#136403=DIRECTION('center_axis',(0.428718122142675,0.311481948263332,-0.848044673146726));
#136404=DIRECTION('ref_axis',(0.892441805934785,6.84549135789276E-16,0.451162523953242));
#136405=DIRECTION('center_axis',(0.404512555980279,0.293895562536812,-0.866022511471539));
#136406=DIRECTION('ref_axis',(0.703251077798178,0.505408667887383,0.500000000000001));
#136407=DIRECTION('center_axis',(-0.404512560891349,-0.293895578599947,
0.86602250372639));
#136408=DIRECTION('ref_axis',(-0.906035256115544,1.03179550260572E-15,-0.423202214875631));
#136409=DIRECTION('center_axis',(0.428718110387558,0.311481908455336,-0.848044693710623));
#136410=DIRECTION('ref_axis',(0.688740099740287,0.494795562231826,0.529919264233176));
#136411=DIRECTION('center_axis',(0.428718069290549,0.3114819098639,-0.848044713969329));
#136412=DIRECTION('ref_axis',(0.892441837073392,2.99591639139466E-15,0.451162462358151));
#136413=DIRECTION('center_axis',(-0.809016994374931,-0.587785252292496,
-4.1044824792529E-15));
#136414=DIRECTION('ref_axis',(-0.587785252292496,0.809016994374931,6.82961998416073E-15));
#136415=DIRECTION('center_axis',(0.809016994374931,0.587785252292496,4.1044824792529E-15));
#136416=DIRECTION('ref_axis',(0.587785252292496,-0.809016994374931,-6.82961998416073E-15));
#136417=DIRECTION('center_axis',(-0.809016994374943,-0.58778525229248,-4.21840575002204E-15));
#136418=DIRECTION('ref_axis',(-0.58778525229248,0.809016994374943,6.8296199841606E-15));
#136419=DIRECTION('center_axis',(-0.809016994374931,-0.587785252292496,
1.04327345066442E-13));
#136420=DIRECTION('ref_axis',(-0.587785252292496,0.809016994374931,6.82961998416073E-15));
#136421=DIRECTION('center_axis',(-0.809016994374943,-0.58778525229248,-4.21840575002204E-15));
#136422=DIRECTION('ref_axis',(-0.58778525229248,0.809016994374943,6.8296199841606E-15));
#136423=DIRECTION('center_axis',(0.700618669264079,0.509071851162291,0.499979330205589));
#136424=DIRECTION('ref_axis',(-0.403924952195115,-0.294660197714492,0.866036951219191));
#136425=DIRECTION('center_axis',(-0.404512670528659,-0.293895658256103,
-0.866022425483304));
#136426=DIRECTION('ref_axis',(0.906035197473506,2.60041954384793E-15,-0.423202340422576));
#136427=DIRECTION('center_axis',(-0.404512677788203,-0.293895663530555,
-0.866022420302472));
#136428=DIRECTION('ref_axis',(0.587785252293442,-0.809016994374244,-6.11933949130544E-13));
#136429=DIRECTION('center_axis',(0.371576139138171,0.334568658444613,-0.866022508720035));
#136430=DIRECTION('ref_axis',(-0.669130606363659,0.743144825473072,-3.70220040960197E-12));
#136431=DIRECTION('center_axis',(0.643597063368372,0.579456972966985,-0.500012436348884));
#136432=DIRECTION('ref_axis',(0.370919252678232,0.335308969594947,0.866017784402721));
#136433=DIRECTION('center_axis',(-0.37157614556582,-0.334568664232125,0.866022503726307));
#136434=DIRECTION('ref_axis',(-0.918982183096524,-2.90533283465756E-16,
-0.394299058014532));
#136435=DIRECTION('center_axis',(-0.743144825477379,-0.669130606358875,
-4.67251405070161E-15));
#136436=DIRECTION('ref_axis',(-0.669130606358875,0.743144825477379,6.82961998416085E-15));
#136437=DIRECTION('center_axis',(0.743144825477389,0.669130606358864,4.7771614063965E-15));
#136438=DIRECTION('ref_axis',(0.669130606358864,-0.743144825477389,-6.82961998416066E-15));
#136439=DIRECTION('center_axis',(0.743144825477406,0.669130606358845,-3.59306599589465E-14));
#136440=DIRECTION('ref_axis',(0.669130606358845,-0.743144825477406,-6.82961998416065E-15));
#136441=DIRECTION('center_axis',(0.743144825477389,0.669130606358864,4.7771614063965E-15));
#136442=DIRECTION('ref_axis',(0.669130606358864,-0.743144825477389,-6.82961998416066E-15));
#136443=DIRECTION('center_axis',(-0.743144825477382,-0.669130606358872,
-4.67251405070159E-15));
#136444=DIRECTION('ref_axis',(-0.669130606358872,0.743144825477382,6.82961998416048E-15));
#136445=DIRECTION('center_axis',(0.393810436983645,0.354588510146755,0.848045003637575));
#136446=DIRECTION('ref_axis',(-0.90697822335776,-4.43466984905637E-15,0.421177518814575));
#136447=DIRECTION('center_axis',(-0.371576246276111,-0.33456875491203,-0.866022425483295));
#136448=DIRECTION('ref_axis',(0.918982131463648,-8.42496017976876E-16,-0.394299178353862));
#136449=DIRECTION('center_axis',(-0.393810401512578,-0.354588507305327,
-0.848045021297503));
#136450=DIRECTION('ref_axis',(-0.627330796743312,-0.570650194823359,0.529919264233208));
#136451=DIRECTION('center_axis',(0.393810395274833,0.354588472591972,0.84804503870866));
#136452=DIRECTION('ref_axis',(-0.906978247051303,2.81492198842025E-15,0.421177467792077));
#136453=DIRECTION('center_axis',(-0.371576249533521,-0.334568771995624,
-0.866022417485796));
#136454=DIRECTION('ref_axis',(-0.640529840772685,-0.582856348579827,0.499999999999909));
#136455=DIRECTION('center_axis',(-0.643614221961003,-0.579466481046856,
-0.499979330205465));
#136456=DIRECTION('ref_axis',(0.372201885192739,0.33383492295115,-0.866036951219271));
#136457=DIRECTION('center_axis',(0.669310796197597,-0.742982542253409,-5.18821936272801E-15));
#136458=DIRECTION('ref_axis',(-0.742982542253409,-0.669310796197597,-3.41480999208022E-15));
#136459=DIRECTION('center_axis',(0.743144825477389,0.669130606358864,4.7771614063965E-15));
#136460=DIRECTION('ref_axis',(0.669130606358864,-0.743144825477389,-6.82961998416066E-15));
#136461=DIRECTION('center_axis',(-0.743144825477379,-0.669130606358875,
-4.67251405070161E-15));
#136462=DIRECTION('ref_axis',(-0.669130606358875,0.743144825477379,6.82961998416085E-15));
#136463=DIRECTION('center_axis',(-2.45464262584879E-16,-7.07718757997909E-15,
1.));
#136464=DIRECTION('ref_axis',(-1.,1.60344088833289E-30,-2.46820266164289E-16));
#136465=DIRECTION('center_axis',(0.668950377172438,-0.743307065001304,-5.19048549296463E-15));
#136466=DIRECTION('ref_axis',(-0.743307065001304,-0.668950377172438,-3.41480999208024E-15));
#136467=DIRECTION('center_axis',(-0.39381078147567,-0.354588820328842,0.84804471396933));
#136468=DIRECTION('ref_axis',(-0.906978027661858,9.58633533089459E-18,-0.421177940232637));
#136469=DIRECTION('center_axis',(-0.393810395274846,-0.354588472591984,
-0.848045038708649));
#136470=DIRECTION('ref_axis',(0.906978247051294,3.98971491588805E-15,-0.421177467792096));
#136471=DIRECTION('center_axis',(-0.393810822585816,-0.354588823412929,
0.848044693589269));
#136472=DIRECTION('ref_axis',(0.627180210728517,0.570815694129948,0.529919264233221));
#136473=DIRECTION('center_axis',(-0.393810830024562,-0.354588864042309,
0.848044673146734));
#136474=DIRECTION('ref_axis',(-0.906978000082632,3.09313791198912E-15,-0.421177999622617));
#136475=DIRECTION('center_axis',(0.393810401584693,0.354588507461832,0.848045021198576));
#136476=DIRECTION('ref_axis',(-0.633098037503341,-0.564245025059131,0.529919264233184));
#136477=DIRECTION('center_axis',(-0.393810436983627,-0.354588510146739,
-0.84804500363759));
#136478=DIRECTION('ref_axis',(0.906978223357771,-2.42620968147434E-15,-0.421177518814551));
#136479=DIRECTION('center_axis',(0.669322449283885,-0.742972044483923,-9.21213603482361E-15));
#136480=DIRECTION('ref_axis',(-0.742972044483923,-0.669322449283885,-3.41480999208054E-15));
#136481=DIRECTION('center_axis',(-0.743144825477406,-0.669130606358845,
-4.6725140507014E-15));
#136482=DIRECTION('ref_axis',(-0.669130606358845,0.743144825477406,6.82961998416065E-15));
#136483=DIRECTION('center_axis',(-2.45464262584879E-16,-7.07718757997909E-15,
1.));
#136484=DIRECTION('ref_axis',(-1.,1.70692667996567E-30,-2.477357166746E-16));
#136485=DIRECTION('center_axis',(0.668938718831625,-0.743317556935059,-5.19055875774645E-15));
#136486=DIRECTION('ref_axis',(-0.743317556935059,-0.668938718831625,-3.41480999208048E-15));
#136487=DIRECTION('center_axis',(-0.743144825477389,-0.669130606358864,
-4.7771614063965E-15));
#136488=DIRECTION('ref_axis',(-0.669130606358865,0.743144825477389,6.82961998416053E-15));
#136489=DIRECTION('center_axis',(-0.643556859036855,-0.579501624400643,
0.500012436348971));
#136490=DIRECTION('ref_axis',(-0.372243731528579,-0.333837986808177,-0.866017784402574));
#136491=DIRECTION('center_axis',(0.393810830024499,0.354588864042367,-0.848044673146739));
#136492=DIRECTION('ref_axis',(0.906978000082658,2.87858588363672E-16,0.421177999622561));
#136493=DIRECTION('center_axis',(0.371576142364791,0.334568647738853,-0.866022511471553));
#136494=DIRECTION('ref_axis',(0.646569003435637,0.576149740776005,0.499999999999988));
#136495=DIRECTION('center_axis',(-0.371576145565792,-0.334568664232036,
0.866022503726353));
#136496=DIRECTION('ref_axis',(-0.918982183096542,-3.10377123333878E-15,
-0.39429905801449));
#136497=DIRECTION('center_axis',(0.393810822485845,0.354588823233822,-0.848044693710583));
#136498=DIRECTION('ref_axis',(0.633246889646911,0.564077964599757,0.529919264233249));
#136499=DIRECTION('center_axis',(0.393810781475714,0.354588820328819,-0.848044713969319));
#136500=DIRECTION('ref_axis',(0.906978027661838,-3.63667371350487E-15,0.421177940232679));
#136501=DIRECTION('center_axis',(-0.743144825477406,-0.669130606358845,
-4.52756880603493E-14));
#136502=DIRECTION('ref_axis',(-0.669130606358845,0.743144825477406,6.82961998416065E-15));
#136503=DIRECTION('center_axis',(0.743144825477379,0.669130606358875,4.67251405070161E-15));
#136504=DIRECTION('ref_axis',(0.669130606358875,-0.743144825477379,-6.82961998416085E-15));
#136505=DIRECTION('center_axis',(-0.743144825477389,-0.669130606358864,
-4.7771614063965E-15));
#136506=DIRECTION('ref_axis',(-0.669130606358865,0.743144825477389,6.82961998416075E-15));
#136507=DIRECTION('center_axis',(-0.743144825477406,-0.669130606358845,
-4.52756880603471E-14));
#136508=DIRECTION('ref_axis',(-0.669130606358845,0.743144825477406,6.82961998416065E-15));
#136509=DIRECTION('center_axis',(-0.743144825477389,-0.669130606358864,
-4.7771614063965E-15));
#136510=DIRECTION('ref_axis',(-0.669130606358865,0.743144825477389,6.82961998416075E-15));
#136511=DIRECTION('center_axis',(0.643568108592016,0.579517695131662,0.499979330205341));
#136512=DIRECTION('ref_axis',(-0.37091183139934,-0.335267672838718,0.866036951219345));
#136513=DIRECTION('center_axis',(-0.37157624627613,-0.33456875491202,-0.866022425483291));
#136514=DIRECTION('ref_axis',(0.91898213146364,-2.37633339499038E-15,-0.39429917835388));
#136515=DIRECTION('center_axis',(-0.371576252942618,-0.334568760914637,
-0.866022420303983));
#136516=DIRECTION('ref_axis',(0.669130606365272,-0.743144825471619,-4.92606829050724E-12));
#136517=DIRECTION('center_axis',(0.334568658444856,0.371576139138533,-0.866022508719786));
#136518=DIRECTION('ref_axis',(-0.743144825477019,0.669130606359275,3.84644198394791E-13));
#136519=DIRECTION('center_axis',(0.579501624400154,0.643556859037784,-0.500012436348342));
#136520=DIRECTION('ref_axis',(0.333837986840269,0.372243731498863,0.866017784402976));
#136521=DIRECTION('center_axis',(-0.3345686642321,-0.371576145565845,0.866022503726305));
#136522=DIRECTION('ref_axis',(-2.10155353069294E-16,-0.918982183096514,
-0.394299058014555));
#136523=DIRECTION('center_axis',(-0.669130606358875,-0.743144825477379,
-5.18935258042421E-15));
#136524=DIRECTION('ref_axis',(-0.743144825477379,0.669130606358875,3.41480999208015E-15));
#136525=DIRECTION('center_axis',(0.669130606358852,0.7431448254774,5.28357748271718E-15));
#136526=DIRECTION('ref_axis',(0.7431448254774,-0.669130606358852,-3.41480999208033E-15));
#136527=DIRECTION('center_axis',(0.669130606358845,0.743144825477406,4.1748614670039E-14));
#136528=DIRECTION('ref_axis',(0.743144825477406,-0.669130606358845,-3.41480999208033E-15));
#136529=DIRECTION('center_axis',(0.669130606358852,0.7431448254774,5.28357748271718E-15));
#136530=DIRECTION('ref_axis',(0.7431448254774,-0.669130606358852,-3.41480999208033E-15));
#136531=DIRECTION('center_axis',(-0.669130606358845,-0.743144825477406,
-5.1893525804244E-15));
#136532=DIRECTION('ref_axis',(-0.743144825477406,0.669130606358845,3.41480999208033E-15));
#136533=DIRECTION('center_axis',(0.354588510146745,0.393810436983621,0.848045003637591));
#136534=DIRECTION('ref_axis',(2.48577593066859E-15,-0.906978223357774,0.421177518814545));
#136535=DIRECTION('center_axis',(-0.334568754912041,-0.371576246276141,
-0.866022425483277));
#136536=DIRECTION('ref_axis',(-3.67049197560442E-15,0.918982131463634,-0.394299178353895));
#136537=DIRECTION('center_axis',(-0.354588475162944,-0.393810430453691,
-0.848045021297511));
#136538=DIRECTION('ref_axis',(-0.564245025068804,-0.633098037494702,0.529919264233205));
#136539=DIRECTION('center_axis',(0.354588472592002,0.393810395274854,0.848045038708637));
#136540=DIRECTION('ref_axis',(-2.96450180524908E-15,-0.906978247051289,
0.421177467792107));
#136541=DIRECTION('center_axis',(-0.334568756368592,-0.371576263604271,
-0.86602241748575));
#136542=DIRECTION('ref_axis',(-0.57609587287649,-0.646617000437385,0.500000000000034));
#136543=DIRECTION('center_axis',(-0.579517695132434,-0.643568108591643,
-0.499979330204926));
#136544=DIRECTION('ref_axis',(0.335267672834376,0.370911831402694,-0.86603695121959));
#136545=DIRECTION('center_axis',(0.743307065001336,-0.668950377172403,-4.67125551701904E-15));
#136546=DIRECTION('ref_axis',(-0.668950377172402,-0.743307065001336,-6.82961998416069E-15));
#136547=DIRECTION('center_axis',(0.669130606358852,0.7431448254774,5.28357748271718E-15));
#136548=DIRECTION('ref_axis',(0.7431448254774,-0.669130606358852,-3.41480999208033E-15));
#136549=DIRECTION('center_axis',(-0.669130606358872,-0.743144825477382,
-5.18935258042423E-15));
#136550=DIRECTION('ref_axis',(-0.743144825477382,0.669130606358872,3.41480999208052E-15));
#136551=DIRECTION('center_axis',(-2.35041809182734E-16,-7.08761003338124E-15,
1.));
#136552=DIRECTION('ref_axis',(-1.,1.60344088833289E-30,-2.32716250954901E-16));
#136553=DIRECTION('center_axis',(0.742982542253406,-0.669310796197601,-4.67377230962033E-15));
#136554=DIRECTION('ref_axis',(-0.669310796197601,-0.742982542253406,-6.82961998416052E-15));
#136555=DIRECTION('center_axis',(-0.35458882032884,-0.393810781475749,0.848044713969294));
#136556=DIRECTION('ref_axis',(-2.33925611613224E-15,-0.906978027661818,
-0.421177940232722));
#136557=DIRECTION('center_axis',(-0.354588472592004,-0.393810395274856,
-0.848045038708635));
#136558=DIRECTION('ref_axis',(1.94126359720515E-15,0.906978247051288,-0.421177467792109));
#136559=DIRECTION('center_axis',(-0.354588860888781,-0.393810788842403,
0.848044693589271));
#136560=DIRECTION('ref_axis',(0.564077964581017,0.63324688966366,0.529919264233183));
#136561=DIRECTION('center_axis',(-0.354588864042363,-0.393810830024504,
0.848044673146738));
#136562=DIRECTION('ref_axis',(-8.09796269128675E-16,-0.906978000082656,
-0.421177999622565));
#136563=DIRECTION('center_axis',(0.354588475230927,0.393810430605494,0.848045021198593));
#136564=DIRECTION('ref_axis',(-0.570650194812903,-0.627330796752771,0.529919264233269));
#136565=DIRECTION('center_axis',(-0.354588510146774,-0.393810436983654,
-0.848045003637564));
#136566=DIRECTION('ref_axis',(3.03817507168769E-15,0.906978223357754,-0.421177518814587));
#136567=DIRECTION('center_axis',(0.743317556935089,-0.668938718831591,-6.07340514377938E-16));
#136568=DIRECTION('ref_axis',(-0.668938718831591,-0.743317556935089,-6.82961998416058E-15));
#136569=DIRECTION('center_axis',(-0.669130606358845,-0.743144825477406,
-5.1893525804244E-15));
#136570=DIRECTION('ref_axis',(-0.743144825477406,0.669130606358845,3.41480999208033E-15));
#136571=DIRECTION('center_axis',(-2.35041809182734E-16,-7.08761003338124E-15,
1.));
#136572=DIRECTION('ref_axis',(-1.,1.70692667996567E-30,-2.32721430815534E-16));
#136573=DIRECTION('center_axis',(0.742972044483923,-0.669322449283885,-6.49863705058595E-16));
#136574=DIRECTION('ref_axis',(-0.669322449283885,-0.742972044483923,-6.82961998416067E-15));
#136575=DIRECTION('center_axis',(-0.669130606358852,-0.7431448254774,-5.28357748271718E-15));
#136576=DIRECTION('ref_axis',(-0.7431448254774,0.669130606358852,3.41480999208037E-15));
#136577=DIRECTION('center_axis',(-0.5794569729669,-0.64359706336836,0.500012436348998));
#136578=DIRECTION('ref_axis',(-0.335308969632734,-0.370919252644328,-0.866017784402611));
#136579=DIRECTION('center_axis',(0.354588864042318,0.393810830024554,-0.848044673146734));
#136580=DIRECTION('ref_axis',(-1.8846300391506E-15,0.906978000082635,0.421177999622611));
#136581=DIRECTION('center_axis',(0.334568662774178,0.371576128826869,-0.866022511471576));
#136582=DIRECTION('ref_axis',(0.582802983776954,0.640578396529848,0.499999999999928));
#136583=DIRECTION('center_axis',(-0.334568664232029,-0.371576145565797,
0.866022503726353));
#136584=DIRECTION('ref_axis',(-2.68749946785539E-15,-0.91898218309654,-0.394299058014494));
#136585=DIRECTION('center_axis',(0.354588860816318,0.393810788646376,-0.8480446937106));
#136586=DIRECTION('ref_axis',(0.5708156941274,0.627180210730821,0.52991926423324));
#136587=DIRECTION('center_axis',(0.354588820328778,0.39381078147575,-0.848044713969319));
#136588=DIRECTION('ref_axis',(2.773318553842E-15,0.906978027661822,0.421177940232713));
#136589=DIRECTION('center_axis',(-0.669130606358845,-0.743144825477406,
3.54138214292235E-14));
#136590=DIRECTION('ref_axis',(-0.743144825477406,0.669130606358845,3.41480999208033E-15));
#136591=DIRECTION('center_axis',(0.669130606358872,0.743144825477382,5.18935258042423E-15));
#136592=DIRECTION('ref_axis',(0.743144825477382,-0.669130606358872,-3.41480999208052E-15));
#136593=DIRECTION('center_axis',(-0.669130606358852,-0.7431448254774,-5.28357748271718E-15));
#136594=DIRECTION('ref_axis',(-0.7431448254774,0.669130606358852,3.41480999208037E-15));
#136595=DIRECTION('center_axis',(-0.669130606358845,-0.743144825477406,
3.13699095091902E-14));
#136596=DIRECTION('ref_axis',(-0.743144825477406,0.669130606358845,3.41480999208033E-15));
#136597=DIRECTION('center_axis',(-0.669130606358852,-0.7431448254774,-5.28357748271718E-15));
#136598=DIRECTION('ref_axis',(-0.7431448254774,0.669130606358852,3.41480999208037E-15));
#136599=DIRECTION('center_axis',(0.579466481046767,0.643614221961237,0.499979330205268));
#136600=DIRECTION('ref_axis',(-0.333834922934168,-0.372201885207748,0.866036951219367));
#136601=DIRECTION('center_axis',(-0.334568754912033,-0.371576246276132,
-0.866022425483285));
#136602=DIRECTION('ref_axis',(-2.55402912997765E-15,0.918982131463639,-0.394299178353883));
#136603=DIRECTION('center_axis',(-0.334568760920321,-0.371576252949017,
-0.866022420299042));
#136604=DIRECTION('ref_axis',(0.743144825474438,-0.669130606362141,2.55700971598187E-12));
#136605=DIRECTION('center_axis',(0.29389557351548,0.404512553893185,-0.866022508720657));
#136606=DIRECTION('ref_axis',(-0.809016994376333,0.587785252290566,-1.38996426237733E-12));
#136607=DIRECTION('center_axis',(0.509057044367788,0.700605801485607,-0.500012436349579));
#136608=DIRECTION('ref_axis',(0.293099122190702,0.405100113144966,0.866017784402246));
#136609=DIRECTION('center_axis',(-0.293895578600024,-0.40451256089147,0.866022503726307));
#136610=DIRECTION('ref_axis',(2.32982689944053E-15,-0.90603525611548,-0.423202214875768));
#136611=DIRECTION('center_axis',(-0.58778525229247,-0.80901699437495,-5.6493354773342E-15));
#136612=DIRECTION('ref_axis',(-0.80901699437495,0.58778525229247,3.41480999208022E-15));
#136613=DIRECTION('center_axis',(0.587785252292466,0.809016994374953,5.73210557847754E-15));
#136614=DIRECTION('ref_axis',(0.809016994374953,-0.587785252292466,-3.41480999208033E-15));
#136615=DIRECTION('center_axis',(0.58778525229247,0.80901699437495,5.6493354773342E-15));
#136616=DIRECTION('ref_axis',(0.80901699437495,-0.58778525229247,-3.41480999208022E-15));
#136617=DIRECTION('center_axis',(0.587785252292466,0.809016994374953,5.73210557847754E-15));
#136618=DIRECTION('ref_axis',(0.809016994374953,-0.587785252292466,-3.41480999208033E-15));
#136619=DIRECTION('center_axis',(-0.58778525229247,-0.80901699437495,-5.6493354773342E-15));
#136620=DIRECTION('ref_axis',(-0.80901699437495,0.58778525229247,3.41480999208022E-15));
#136621=DIRECTION('center_axis',(0.311481637390299,0.428717694262763,0.848045003637589));
#136622=DIRECTION('ref_axis',(1.51664064046204E-16,-0.89244205802627,0.451162025292284));
#136623=DIRECTION('center_axis',(-0.293895658256123,-0.404512670528727,
-0.866022425483265));
#136624=DIRECTION('ref_axis',(-1.09162433120364E-15,0.906035197473472,-0.423202340422648));
#136625=DIRECTION('center_axis',(-0.311481603281241,-0.4287176841114,-0.848045021297516));
#136626=DIRECTION('ref_axis',(-0.494977266824932,-0.68860952558114,0.529919264233183));
#136627=DIRECTION('center_axis',(0.311481604401019,0.428717648856915,0.848045038708656));
#136628=DIRECTION('ref_axis',(-1.55513761614889E-15,-0.89244208477774,0.45116197237529));
#136629=DIRECTION('center_axis',(-0.293895657890896,-0.404512687915994,
-0.866022417485746));
#136630=DIRECTION('ref_axis',(-0.505350078025385,-0.703293181141193,0.500000000000038));
#136631=DIRECTION('center_axis',(-0.509071851163456,-0.700618669263731,
-0.49997933020489));
#136632=DIRECTION('ref_axis',(0.294660197697665,0.403924952206488,-0.866036951219611));
#136633=DIRECTION('center_axis',(0.809159506053914,-0.587589051772227,-4.10311241834253E-15));
#136634=DIRECTION('ref_axis',(-0.587589051772227,-0.809159506053914,-6.82961998416088E-15));
#136635=DIRECTION('center_axis',(0.587785252292466,0.809016994374953,5.73210557847754E-15));
#136636=DIRECTION('ref_axis',(0.809016994374953,-0.587785252292466,-3.41480999208033E-15));
#136637=DIRECTION('center_axis',(-0.58778525229247,-0.80901699437495,-5.6493354773342E-15));
#136638=DIRECTION('ref_axis',(-0.80901699437495,0.58778525229247,3.41480999208022E-15));
#136639=DIRECTION('center_axis',(-2.23587008033241E-16,-7.09688594845552E-15,
1.));
#136640=DIRECTION('ref_axis',(-1.,1.60344088833289E-30,-2.25664243350207E-16));
#136641=DIRECTION('center_axis',(0.808874435122379,-0.587981418248444,-4.10585229880193E-15));
#136642=DIRECTION('ref_axis',(-0.587981418248444,-0.808874435122379,-6.82961998416087E-15));
#136643=DIRECTION('center_axis',(-0.311481909863932,-0.428718069290528,
0.848044713969328));
#136644=DIRECTION('ref_axis',(3.08013998868981E-15,-0.892441837073401,-0.451162462358132));
#136645=DIRECTION('center_axis',(-0.311481604401018,-0.428717648856992,
-0.848045038708618));
#136646=DIRECTION('ref_axis',(3.62313198634112E-15,0.892442084777698,-0.451161972375371));
#136647=DIRECTION('center_axis',(-0.311481949432504,-0.428718080855936,
0.848044693589277));
#136648=DIRECTION('ref_axis',(0.494795562236623,0.688740099736818,0.529919264233205));
#136649=DIRECTION('center_axis',(-0.311481948263276,-0.428718122142692,
0.848044673146738));
#136650=DIRECTION('ref_axis',(-3.57201939485921E-16,-0.892441805934781,
-0.451162523953251));
#136651=DIRECTION('center_axis',(0.311481603328271,0.428717684272931,0.848045021198583));
#136652=DIRECTION('ref_axis',(-0.501950189201534,-0.683543400930078,0.52991926423323));
#136653=DIRECTION('center_axis',(-0.311481637390294,-0.428717694262756,
-0.848045003637594));
#136654=DIRECTION('ref_axis',(7.82282120695661E-16,0.892442058026274,-0.451162025292277));
#136655=DIRECTION('center_axis',(0.809168721883286,-0.587576360591345,8.00410915583402E-15));
#136656=DIRECTION('ref_axis',(-0.587576360591345,-0.809168721883286,-6.82961998416048E-15));
#136657=DIRECTION('center_axis',(-0.58778525229247,-0.80901699437495,-5.6493354773342E-15));
#136658=DIRECTION('ref_axis',(-0.80901699437495,0.58778525229247,3.41480999208022E-15));
#136659=DIRECTION('center_axis',(-2.23587008033241E-16,-7.09688594845552E-15,
1.));
#136660=DIRECTION('ref_axis',(-1.,1.70692667996567E-30,-2.25214287886E-16));
#136661=DIRECTION('center_axis',(0.808865212939984,-0.587994104813606,-4.10594088861296E-15));
#136662=DIRECTION('ref_axis',(-0.587994104813606,-0.808865212939984,-6.82961998416048E-15));
#136663=DIRECTION('center_axis',(-0.587785252292466,-0.809016994374953,
-5.73210557847754E-15));
#136664=DIRECTION('ref_axis',(-0.809016994374953,0.587785252292466,3.41480999208036E-15));
#136665=DIRECTION('center_axis',(-0.509008435042705,-0.700641118228387,
0.50001243634839));
#136666=DIRECTION('ref_axis',(-0.294700492572351,-0.403936649458133,-0.866017784402925));
#136667=DIRECTION('center_axis',(0.31148194826325,0.428718122142734,-0.848044673146726));
#136668=DIRECTION('ref_axis',(-2.26428405615115E-15,0.89244180593476,0.451162523953291));
#136669=DIRECTION('center_axis',(0.293895578898316,0.404512544092887,-0.866022511471569));
#136670=DIRECTION('ref_axis',(0.512651652655376,0.697988741334513,0.499999999999974));
#136671=DIRECTION('center_axis',(-0.293895578599974,-0.404512560891429,
0.866022503726344));
#136672=DIRECTION('ref_axis',(-1.18885620953251E-15,-0.906035256115503,
-0.423202214875719));
#136673=DIRECTION('center_axis',(0.311481949380855,0.428718080653442,-0.848044693710615));
#136674=DIRECTION('ref_axis',(0.502130522406322,0.683410939232379,0.529919264233214));
#136675=DIRECTION('center_axis',(0.311481909863867,0.428718069290587,-0.848044713969322));
#136676=DIRECTION('ref_axis',(1.35835357911667E-15,0.892441837073374,0.451162462358185));
#136677=DIRECTION('center_axis',(-0.58778525229247,-0.80901699437495,-5.6493354773342E-15));
#136678=DIRECTION('ref_axis',(-0.80901699437495,0.58778525229247,3.41480999208022E-15));
#136679=DIRECTION('center_axis',(0.587785252292496,0.809016994374931,5.64933547733406E-15));
#136680=DIRECTION('ref_axis',(0.809016994374931,-0.587785252292496,-3.41480999208037E-15));
#136681=DIRECTION('center_axis',(-0.587785252292466,-0.809016994374953,
-5.73210557847754E-15));
#136682=DIRECTION('ref_axis',(-0.809016994374953,0.587785252292466,3.41480999208036E-15));
#136683=DIRECTION('center_axis',(-0.58778525229247,-0.80901699437495,-1.77367652921915E-14));
#136684=DIRECTION('ref_axis',(-0.80901699437495,0.58778525229247,3.41480999208022E-15));
#136685=DIRECTION('center_axis',(-0.587785252292466,-0.809016994374953,
-5.73210557847754E-15));
#136686=DIRECTION('ref_axis',(-0.809016994374953,0.587785252292466,3.41480999208036E-15));
#136687=DIRECTION('center_axis',(0.509016097474163,0.70065917669004,0.499979330204968));
#136688=DIRECTION('ref_axis',(-0.293100449223401,-0.405058175806119,0.866036951219553));
#136689=DIRECTION('center_axis',(-0.293895658256093,-0.404512670528659,
-0.866022425483307));
#136690=DIRECTION('ref_axis',(3.08674820555281E-15,0.906035197473506,-0.423202340422574));
#136691=DIRECTION('center_axis',(-0.293895663531409,-0.404512677789524,
-0.866022420301566));
#136692=DIRECTION('ref_axis',(0.809016994376599,-0.5877852522902,-1.62599592197905E-12));
#136693=DIRECTION('center_axis',(0.250002507179564,0.433017044454593,-0.866022508723498));
#136694=DIRECTION('ref_axis',(-0.866025403783392,0.500000000001813,1.20201311999016E-12));
#136695=DIRECTION('center_axis',(0.433035128830174,0.749978760162262,-0.500012436349849));
#136696=DIRECTION('ref_axis',(0.249149002239919,0.433518133164162,0.866017784402095));
#136697=DIRECTION('center_axis',(-0.25000251150716,-0.433017051950299,0.866022503726309));
#136698=DIRECTION('ref_axis',(1.53376353322716E-15,-0.894424794863775,-0.447218387740144));
#136699=DIRECTION('center_axis',(-0.500000000000022,-0.866025403784426,
-6.04742307255483E-15));
#136700=DIRECTION('ref_axis',(-0.866025403784426,0.500000000000022,3.41480999208042E-15));
#136701=DIRECTION('center_axis',(0.499999999999992,0.866025403784443,6.1178315259999E-15));
#136702=DIRECTION('ref_axis',(0.866025403784443,-0.499999999999992,-3.41480999208033E-15));
#136703=DIRECTION('center_axis',(0.50000000000001,0.866025403784433,-7.61181689576648E-15));
#136704=DIRECTION('ref_axis',(0.866025403784433,-0.50000000000001,-3.41480999208034E-15));
#136705=DIRECTION('center_axis',(0.499999999999992,0.866025403784443,6.1178315259999E-15));
#136706=DIRECTION('ref_axis',(0.866025403784443,-0.499999999999992,-3.41480999208033E-15));
#136707=DIRECTION('center_axis',(-0.50000000000001,-0.866025403784433,-6.04742307255487E-15));
#136708=DIRECTION('ref_axis',(-0.866025403784433,0.50000000000001,3.41480999208034E-15));
#136709=DIRECTION('center_axis',(0.264962106632875,0.458927830768604,0.848045003637597));
#136710=DIRECTION('ref_axis',(-1.67218023172745E-15,-0.879478602053344,
0.475938429348058));
#136711=DIRECTION('center_axis',(-0.25000257926675,-0.433017169313239,-0.866022425483268));
#136712=DIRECTION('ref_axis',(-1.10825904974603E-15,0.894424730216403,-0.447218517033133));
#136713=DIRECTION('center_axis',(-0.264962073768116,-0.458927817109621,
-0.848045021297512));
#136714=DIRECTION('ref_axis',(-0.420286434051416,-0.736576463611834,0.529919264233175));
#136715=DIRECTION('center_axis',(0.264962078570529,0.458927782163195,0.84804503870865));
#136716=DIRECTION('ref_axis',(-1.38504843431592E-15,-0.879478631391255,
0.475938375135021));
#136717=DIRECTION('center_axis',(-0.250002577085399,-0.433017186567401,
-0.866022417485778));
#136718=DIRECTION('ref_axis',(-0.4290675619629,-0.752263934580973,0.499999999999966));
#136719=DIRECTION('center_axis',(-0.433048509462545,-0.749993105181572,
-0.499979330205131));
#136720=DIRECTION('ref_axis',(0.250824363776163,0.432512586705598,-0.866036951219471));
#136721=DIRECTION('center_axis',(0.866146626230631,-0.499789977759954,-3.49001476137941E-15));
#136722=DIRECTION('ref_axis',(-0.499789977759954,-0.866146626230631,-6.82961998416062E-15));
#136723=DIRECTION('center_axis',(0.499999999999992,0.866025403784443,6.1178315259999E-15));
#136724=DIRECTION('ref_axis',(0.866025403784443,-0.499999999999992,-3.41480999208033E-15));
#136725=DIRECTION('center_axis',(-0.499999999999998,-0.86602540378444,-6.04742307255492E-15));
#136726=DIRECTION('ref_axis',(-0.86602540378444,0.499999999999998,3.41480999208026E-15));
#136727=DIRECTION('center_axis',(-2.11225360334865E-16,-7.10491369633528E-15,
1.));
#136728=DIRECTION('ref_axis',(-1.,1.60344088833289E-30,-2.11560228140819E-16));
#136729=DIRECTION('center_axis',(0.865904130412297,-0.500209992837931,-3.49294771099299E-15));
#136730=DIRECTION('ref_axis',(-0.500209992837931,-0.865904130412297,-6.82961998416051E-15));
#136731=DIRECTION('center_axis',(-0.264962338412774,-0.45892823222322,0.848044713969319));
#136732=DIRECTION('ref_axis',(2.43676345907576E-15,-0.879478359737737,-0.475938877118711));
#136733=DIRECTION('center_axis',(-0.264962078570521,-0.458927782163195,
-0.848045038708653));
#136734=DIRECTION('ref_axis',(1.53522557929348E-15,0.879478631391256,-0.475938375135021));
#136735=DIRECTION('center_axis',(-0.264962376555394,-0.458928247861462,
0.848044693589274));
#136736=DIRECTION('ref_axis',(0.420092076167741,0.736687329153681,0.529919264233235));
#136737=DIRECTION('center_axis',(-0.264962371077221,-0.458928288799658,
0.848044673146736));
#136738=DIRECTION('ref_axis',(1.01699383191385E-17,-0.879478325588507,-0.475938940222416));
#136739=DIRECTION('center_axis',(0.264962073791877,0.458927817278717,0.848045021198581));
#136740=DIRECTION('ref_axis',(-0.42775071226141,-0.732266960578161,0.529919264233221));
#136741=DIRECTION('center_axis',(-0.264962106632886,-0.458927830768637,
-0.848045003637576));
#136742=DIRECTION('ref_axis',(-2.90135607278746E-16,0.879478602053325,-0.475938429348093));
#136743=DIRECTION('center_axis',(0.86615446498511,-0.499776392786171,-3.48991989801451E-15));
#136744=DIRECTION('ref_axis',(-0.499776392786171,-0.86615446498511,-6.82961998416069E-15));
#136745=DIRECTION('center_axis',(-0.50000000000001,-0.866025403784433,-6.04742307255487E-15));
#136746=DIRECTION('ref_axis',(-0.866025403784433,0.50000000000001,3.41480999208034E-15));
#136747=DIRECTION('center_axis',(-2.11225360334865E-16,-7.10491369633528E-15,
1.));
#136748=DIRECTION('ref_axis',(-1.,1.70692667996567E-30,-2.10200002026934E-16));
#136749=DIRECTION('center_axis',(0.865896284857143,-0.500223573885315,2.38376527871029E-14));
#136750=DIRECTION('ref_axis',(-0.500223573885315,-0.865896284857143,-6.82961998416031E-15));
#136751=DIRECTION('center_axis',(-0.499999999999992,-0.866025403784443,
-6.1178315259999E-15));
#136752=DIRECTION('ref_axis',(-0.866025403784443,0.499999999999992,3.41480999208041E-15));
#136753=DIRECTION('center_axis',(-0.432983094186217,-0.750008802379052,
0.500012436348207));
#136754=DIRECTION('ref_axis',(-0.250863215223843,-0.432528431834534,-0.866017784403019));
#136755=DIRECTION('center_axis',(0.264962371077185,0.45892828879969,-0.84804467314673));
#136756=DIRECTION('ref_axis',(-2.01281341115834E-15,0.879478325588492,0.475938940222443));
#136757=DIRECTION('center_axis',(0.250002513555436,0.433017035277449,-0.866022511471551));
#136758=DIRECTION('ref_axis',(0.436883602746975,0.747751775424735,0.499999999999979));
#136759=DIRECTION('center_axis',(-0.250002511507164,-0.433017051950226,
0.866022503726344));
#136760=DIRECTION('ref_axis',(-2.52000272705874E-15,-0.894424794863812,
-0.44721838774007));
#136761=DIRECTION('center_axis',(0.26496237652361,0.458928247655632,-0.848044693710592));
#136762=DIRECTION('ref_axis',(0.427943903597026,0.732154074473812,0.529919264233274));
#136763=DIRECTION('center_axis',(0.264962338412787,0.4589282322232,-0.848044713969326));
#136764=DIRECTION('ref_axis',(-1.36968032163284E-15,0.879478359737747,0.475938877118692));
#136765=DIRECTION('center_axis',(-0.50000000000001,-0.866025403784433,-6.70236582766912E-14));
#136766=DIRECTION('ref_axis',(-0.866025403784433,0.50000000000001,3.41480999208034E-15));
#136767=DIRECTION('center_axis',(0.499999999999998,0.86602540378444,6.04742307255492E-15));
#136768=DIRECTION('ref_axis',(0.86602540378444,-0.499999999999998,-3.41480999208026E-15));
#136769=DIRECTION('center_axis',(-0.499999999999992,-0.866025403784443,
-6.1178315259999E-15));
#136770=DIRECTION('ref_axis',(-0.866025403784443,0.499999999999992,3.41480999208041E-15));
#136771=DIRECTION('center_axis',(-0.50000000000001,-0.866025403784433,2.12710568640878E-14));
#136772=DIRECTION('ref_axis',(-0.866025403784433,0.50000000000001,3.41480999208034E-15));
#136773=DIRECTION('center_axis',(-0.499999999999992,-0.866025403784443,
-6.1178315259999E-15));
#136774=DIRECTION('ref_axis',(-0.866025403784443,0.499999999999992,3.41480999208041E-15));
#136775=DIRECTION('center_axis',(0.432988827019022,0.750027562856532,0.499979330204942));
#136776=DIRECTION('ref_axis',(-0.249154705652333,-0.433476564272626,0.866036951219576));
#136777=DIRECTION('center_axis',(-0.250002579266693,-0.43301716931316,-0.866022425483324));
#136778=DIRECTION('ref_axis',(-2.14154226504039E-15,0.894424730216448,-0.447218517033044));
#136779=DIRECTION('center_axis',(-0.250002583752831,-0.433017177083424,
-0.866022420303084));
#136780=DIRECTION('ref_axis',(0.866025403788155,-0.499999999993563,-4.2922795574701E-12));
#136781=DIRECTION('center_axis',(0.203370361062878,0.456777309669372,-0.866022508721549));
#136782=DIRECTION('ref_axis',(-0.913545457643545,0.40673664307368,-1.36373852159054E-12));
#136783=DIRECTION('center_axis',(0.352268789801635,0.791134794600313,-0.500012436349749));
#136784=DIRECTION('ref_axis',(0.202469153692936,0.457186437793193,0.866017784402166));
#136785=DIRECTION('center_axis',(-0.203370364581913,-0.456777317573281,
0.866022503726305));
#136786=DIRECTION('ref_axis',(-9.65527517661163E-16,-0.884507036382094,
-0.466526850878452));
#136787=DIRECTION('center_axis',(-0.406736643075807,-0.913545457642598,
-6.37925383508808E-15));
#136788=DIRECTION('ref_axis',(-0.913545457642598,0.406736643075807,3.4148099920803E-15));
#136789=DIRECTION('center_axis',(0.406736643075792,0.913545457642605,6.43652923108485E-15));
#136790=DIRECTION('ref_axis',(0.913545457642605,-0.406736643075792,-3.41480999208033E-15));
#136791=DIRECTION('center_axis',(0.406736643075807,0.913545457642598,6.37925383508808E-15));
#136792=DIRECTION('ref_axis',(0.913545457642598,-0.406736643075807,-3.4148099920803E-15));
#136793=DIRECTION('center_axis',(0.406736643075792,0.913545457642605,6.43652923108485E-15));
#136794=DIRECTION('ref_axis',(0.913545457642605,-0.406736643075792,-3.41480999208033E-15));
#136795=DIRECTION('center_axis',(-0.406736643075751,-0.913545457642623,
-6.37925383508826E-15));
#136796=DIRECTION('ref_axis',(-0.913545457642623,0.406736643075751,3.41480999208029E-15));
#136797=DIRECTION('center_axis',(0.215539595588322,0.4841098579238,0.848045003637555));
#136798=DIRECTION('ref_axis',(2.30068443353737E-15,-0.868458021515977,0.495762710240045));
#136799=DIRECTION('center_axis',(-0.20337041970245,-0.456777441376071,-0.866022425483301));
#136800=DIRECTION('ref_axis',(-1.81723778193288E-15,0.884506966812061,-0.466526982779054));
#136801=DIRECTION('center_axis',(-0.215539564333521,-0.484109840903322,
-0.848045021297499));
#136802=DIRECTION('ref_axis',(-0.340990855200675,-0.776473315744986,0.52991926423324));
#136803=DIRECTION('center_axis',(0.215539572760323,0.484109806651273,0.848045038708655));
#136804=DIRECTION('ref_axis',(-1.36803287013151E-15,-0.868458052949966,
0.49576265517519));
#136805=DIRECTION('center_axis',(-0.203370415729637,-0.456777458307746,
-0.866022417485754));
#136806=DIRECTION('ref_axis',(-0.348084091918547,-0.792992726923284,0.500000000000014));
#136807=DIRECTION('center_axis',(-0.352280597671235,-0.791150459692768,
-0.499979330205079));
#136808=DIRECTION('ref_axis',(0.204240445642775,0.456361522793153,-0.866036951219493));
#136809=DIRECTION('center_axis',(0.913644062717554,-0.406515100163527,2.21206872242239E-14));
#136810=DIRECTION('ref_axis',(-0.406515100163527,-0.913644062717554,-6.82961998416096E-15));
#136811=DIRECTION('center_axis',(0.406736643075792,0.913545457642605,6.43652923108485E-15));
#136812=DIRECTION('ref_axis',(0.913545457642605,-0.406736643075792,-3.41480999208033E-15));
#136813=DIRECTION('center_axis',(-0.406736643075807,-0.913545457642598,
-6.37925383508808E-15));
#136814=DIRECTION('ref_axis',(-0.913545457642598,0.406736643075807,3.4148099920803E-15));
#136815=DIRECTION('center_axis',(-1.98092302886629E-16,-7.11160532333483E-15,
1.));
#136816=DIRECTION('ref_axis',(-1.,1.60344088833289E-30,-1.97456212931431E-16));
#136817=DIRECTION('center_axis',(0.913446798847323,-0.406958162070229,-2.84177365711621E-15));
#136818=DIRECTION('ref_axis',(-0.406958162070229,-0.913446798847323,-6.82961998416051E-15));
#136819=DIRECTION('center_axis',(-0.215539784135063,-0.484110281406773,
0.848044713969297));
#136820=DIRECTION('ref_axis',(1.36848187759281E-15,-0.868457761888255,-0.495763165045612));
#136821=DIRECTION('center_axis',(-0.215539572760323,-0.484109806651275,
-0.848045038708654));
#136822=DIRECTION('ref_axis',(1.54244339943813E-15,0.868458052949965,-0.495762655175192));
#136823=DIRECTION('center_axis',(-0.215539820432031,-0.484110300947188,
0.848044693589289));
#136824=DIRECTION('ref_axis',(0.340785973391266,0.776563258037815,0.529919264233205));
#136825=DIRECTION('center_axis',(-0.215539810706713,-0.484110341087614,
0.848044673146733));
#136826=DIRECTION('ref_axis',(-2.60145221568461E-16,-0.868457725299267,
-0.495763229140709));
#136827=DIRECTION('center_axis',(0.215539564341324,0.484109841073138,0.848045021198576));
#136828=DIRECTION('ref_axis',(-0.348864709028221,-0.772967650156986,0.529919264233187));
#136829=DIRECTION('center_axis',(-0.215539595588306,-0.484109857923764,
-0.84804500363758));
#136830=DIRECTION('ref_axis',(1.59176767299167E-16,0.868458021515999,-0.495762710240007));
#136831=DIRECTION('center_axis',(0.913650438514074,-0.406500770236713,-2.83857970701369E-15));
#136832=DIRECTION('ref_axis',(-0.406500770236713,-0.913650438514073,-6.82961998416048E-15));
#136833=DIRECTION('center_axis',(-0.406736643075807,-0.913545457642598,
-4.51811735233643E-14));
#136834=DIRECTION('ref_axis',(-0.913545457642598,0.406736643075807,3.41480999208031E-15));
#136835=DIRECTION('center_axis',(-1.98092302886629E-16,-7.11160532333483E-15,
1.));
#136836=DIRECTION('ref_axis',(-1.,1.28019500997425E-30,-1.95185716167867E-16));
#136837=DIRECTION('center_axis',(0.913440415876957,-0.406972488803028,2.21119299742975E-14));
#136838=DIRECTION('ref_axis',(-0.406972488803028,-0.913440415876957,-6.82961998416073E-15));
#136839=DIRECTION('center_axis',(-0.406736643075792,-0.913545457642605,
-6.43652923108485E-15));
#136840=DIRECTION('ref_axis',(-0.913545457642605,0.406736643075792,3.4148099920804E-15));
#136841=DIRECTION('center_axis',(-0.352213899942465,-0.791159233140713,
0.500012436348855));
#136842=DIRECTION('ref_axis',(-0.204277427961246,-0.456381342217048,-0.866017784402667));
#136843=DIRECTION('center_axis',(0.215539810706706,0.484110341087612,-0.848044673146735));
#136844=DIRECTION('ref_axis',(8.90622427310465E-16,0.868457725299268,0.495763229140707));
#136845=DIRECTION('center_axis',(0.203370368364315,0.456777301204695,-0.866022511471566));
#136846=DIRECTION('ref_axis',(0.356328964674119,0.789322284579817,0.49999999999997));
#136847=DIRECTION('center_axis',(-0.203370364581893,-0.456777317573237,
0.866022503726333));
#136848=DIRECTION('ref_axis',(1.98101988738834E-15,-0.884507036382119,-0.466526850878405));
#136849=DIRECTION('center_axis',(0.215539820424864,0.484110300737865,-0.848044693710603));
#136850=DIRECTION('ref_axis',(0.349068641867812,0.772875576441078,0.529919264233178));
#136851=DIRECTION('center_axis',(0.215539784134997,0.484110281406756,-0.848044713969323));
#136852=DIRECTION('ref_axis',(1.51050753005434E-16,0.868457761888269,0.495763165045588));
#136853=DIRECTION('center_axis',(-0.406736643075807,-0.913545457642598,
-1.74906806584517E-14));
#136854=DIRECTION('ref_axis',(-0.913545457642598,0.406736643075807,3.4148099920803E-15));
#136855=DIRECTION('center_axis',(0.406736643075751,0.913545457642623,6.37925383508826E-15));
#136856=DIRECTION('ref_axis',(0.913545457642623,-0.406736643075751,-3.41480999208029E-15));
#136857=DIRECTION('center_axis',(-0.406736643075792,-0.913545457642605,
-6.43652923108485E-15));
#136858=DIRECTION('ref_axis',(-0.913545457642605,0.406736643075792,3.4148099920804E-15));
#136859=DIRECTION('center_axis',(-0.406736643075807,-0.913545457642598,
-3.40697467000007E-14));
#136860=DIRECTION('ref_axis',(-0.913545457642598,0.406736643075807,3.4148099920803E-15));
#136861=DIRECTION('center_axis',(-0.406736643075792,-0.913545457642605,
-6.43652923108485E-15));
#136862=DIRECTION('ref_axis',(-0.913545457642605,0.406736643075792,3.4148099920804E-15));
#136863=DIRECTION('center_axis',(0.352217640366581,0.791178490090709,0.499979330205143));
#136864=DIRECTION('ref_axis',(-0.202479170975218,-0.457145692797927,0.866036951219457));
#136865=DIRECTION('center_axis',(-0.203370419702468,-0.456777441376064,
-0.8660224254833));
#136866=DIRECTION('ref_axis',(-1.18383422398248E-15,0.884506966812064,-0.466526982779048));
#136867=DIRECTION('center_axis',(-0.203370423354184,-0.456777449577961,
-0.866022420299725));
#136868=DIRECTION('ref_axis',(0.913545457639069,-0.406736643083733,5.02660029640274E-12));
#136869=DIRECTION('center_axis',(0.154510046711354,0.475533027091701,-0.866022508720332));
#136870=DIRECTION('ref_axis',(-0.95105651629323,0.309016994380866,3.59292648953259E-12));
#136871=DIRECTION('center_axis',(0.267642920194089,0.823622990673941,-0.500012436348632));
#136872=DIRECTION('ref_axis',(0.153571010675692,0.475845712156948,0.866017784402776));
#136873=DIRECTION('center_axis',(-0.154510049384264,-0.475533035318161,
0.8660225037263));
#136874=DIRECTION('ref_axis',(-1.50358015652835E-15,-0.876548788012424,
-0.481313018974088));
#136875=DIRECTION('center_axis',(-0.309016994374914,-0.951056516295165,
-6.64119215765945E-15));
#136876=DIRECTION('ref_axis',(-0.951056516295164,0.309016994374914,3.41480999208033E-15));
#136877=DIRECTION('center_axis',(0.309016994374938,0.951056516295157,6.68470697498369E-15));
#136878=DIRECTION('ref_axis',(0.951056516295157,-0.309016994374938,-3.41480999208033E-15));
#136879=DIRECTION('center_axis',(0.309016994374914,0.951056516295164,6.70459034366198E-14));
#136880=DIRECTION('ref_axis',(0.951056516295164,-0.309016994374914,-3.41480999208034E-15));
#136881=DIRECTION('center_axis',(0.309016994374938,0.951056516295157,6.68470697498369E-15));
#136882=DIRECTION('ref_axis',(0.951056516295157,-0.309016994374938,-3.41480999208033E-15));
#136883=DIRECTION('center_axis',(-0.30901699437498,-0.951056516295143,-6.64119215765931E-15));
#136884=DIRECTION('ref_axis',(-0.951056516295143,0.30901699437498,3.41480999208042E-15));
#136885=DIRECTION('center_axis',(0.163755587629875,0.503987876168979,0.848045003637588));
#136886=DIRECTION('ref_axis',(-4.64722749497856E-16,-0.859649462041492,
0.510884333691857));
#136887=DIRECTION('center_axis',(-0.154510091261946,-0.475533164204402,
-0.866022425483298));
#136888=DIRECTION('ref_axis',(-5.65902027059014E-17,0.876548714628842,-0.481313152617425));
#136889=DIRECTION('center_axis',(-0.163755558328224,-0.503987855973834,
-0.848045021297519));
#136890=DIRECTION('ref_axis',(-0.257959309140581,-0.807862963764457,0.529919264233168));
#136891=DIRECTION('center_axis',(0.163755570286389,0.503987822791218,0.848045038708646));
#136892=DIRECTION('ref_axis',(-1.41598484853067E-15,-0.859649495083696,
0.510884278092747));
#136893=DIRECTION('center_axis',(-0.154510085548364,-0.475533180625675,
-0.866022417485752));
#136894=DIRECTION('ref_axis',(-0.263286939714892,-0.825033325009111,0.499999999999978));
#136895=DIRECTION('center_axis',(-0.267653025932247,-0.823639804208766,
-0.499979330205016));
#136896=DIRECTION('ref_axis',(0.15541882643971,0.475210466541391,-0.866036951219529));
#136897=DIRECTION('center_axis',(0.951131423661017,-0.308786358060986,-2.15624361371854E-15));
#136898=DIRECTION('ref_axis',(-0.308786358060986,-0.951131423661017,-6.82961998416067E-15));
#136899=DIRECTION('center_axis',(0.309016994374938,0.951056516295157,6.68470697498369E-15));
#136900=DIRECTION('ref_axis',(0.951056516295157,-0.309016994374938,-3.41480999208033E-15));
#136901=DIRECTION('center_axis',(-0.309016994374914,-0.951056516295165,
-6.64119215765945E-15));
#136902=DIRECTION('ref_axis',(-0.951056516295164,0.309016994374914,3.41480999208033E-15));
#136903=DIRECTION('center_axis',(-1.84331724214206E-16,-7.11688751458844E-15,
1.));
#136904=DIRECTION('ref_axis',(-1.,1.20258066624967E-30,-1.83352197722043E-16));
#136905=DIRECTION('center_axis',(0.95098155300316,-0.309247612517378,-2.15946453637244E-15));
#136906=DIRECTION('ref_axis',(-0.309247612517378,-0.95098155300316,-6.82961998416082E-15));
#136907=DIRECTION('center_axis',(-0.163755730877748,-0.503988317040613,
0.848044713969296));
#136908=DIRECTION('ref_axis',(-2.05932374345746E-15,-0.859649189130447,
-0.510884792910658));
#136909=DIRECTION('center_axis',(-0.163755570286382,-0.503987822791197,
-0.848045038708659));
#136910=DIRECTION('ref_axis',(-2.40920520154009E-15,0.859649495083709,-0.510884278092725));
#136911=DIRECTION('center_axis',(-0.163755764928173,-0.503988340269717,
0.848044693589297));
#136912=DIRECTION('ref_axis',(0.257746148181657,0.807930997358076,0.529919264233245));
#136913=DIRECTION('center_axis',(-0.163755751065481,-0.503988379172018,
0.848044673146729));
#136914=DIRECTION('ref_axis',(-1.44619219902002E-15,-0.859649150669456,
-0.510884857627707));
#136915=DIRECTION('center_axis',(0.163755558317298,0.503987856143866,0.84804502119858));
#136916=DIRECTION('ref_axis',(-0.266156471020706,-0.805199544416383,0.529919264233198));
#136917=DIRECTION('center_axis',(-0.163755587629886,-0.503987876169014,
-0.848045003637565));
#136918=DIRECTION('ref_axis',(-1.56939166226977E-15,0.859649462041471,-0.510884333691893));
#136919=DIRECTION('center_axis',(0.951136266645031,-0.308771440182787,1.47141933445522E-14));
#136920=DIRECTION('ref_axis',(-0.308771440182787,-0.951136266645031,-6.82961998416084E-15));
#136921=DIRECTION('center_axis',(-0.309016994374914,-0.951056516295165,
-6.64119215765945E-15));
#136922=DIRECTION('ref_axis',(-0.951056516295164,0.309016994374914,3.41480999208033E-15));
#136923=DIRECTION('center_axis',(-1.84331724214206E-16,-7.11688751458844E-15,
1.));
#136924=DIRECTION('ref_axis',(-1.,1.28019500997425E-30,-1.87678573238334E-16));
#136925=DIRECTION('center_axis',(0.950976702550726,-0.309262527968953,1.4737595640537E-14));
#136926=DIRECTION('ref_axis',(-0.309262527968953,-0.950976702550726,-6.82961998416076E-15));
#136927=DIRECTION('center_axis',(-0.309016994374938,-0.951056516295157,
-6.68470697498369E-15));
#136928=DIRECTION('ref_axis',(-0.951056516295156,0.309016994374938,3.41480999208031E-15));
#136929=DIRECTION('center_axis',(-0.267585776506164,-0.823641557784294,
0.500012436347593));
#136930=DIRECTION('ref_axis',(-0.155453534446431,-0.475234043104139,-0.866017784403418));
#136931=DIRECTION('center_axis',(0.163755751065396,0.503988379172029,-0.848044673146739));
#136932=DIRECTION('ref_axis',(8.46156807197952E-16,0.859649150669455,0.51088485762771));
#136933=DIRECTION('center_axis',(0.154510054856538,0.475533019434788,-0.866022511471534));
#136934=DIRECTION('ref_axis',(0.271870311892821,0.822244813611669,0.500000000000011));
#136935=DIRECTION('center_axis',(-0.154510049384232,-0.47553303531805,0.866022503726367));
#136936=DIRECTION('ref_axis',(1.97566536568584E-15,-0.876548788012487,-0.481313018973972));
#136937=DIRECTION('center_axis',(0.163755764947861,0.503988340059225,-0.84804469371059));
#136938=DIRECTION('ref_axis',(0.266368910994597,0.805129291884236,0.52991926423328));
#136939=DIRECTION('center_axis',(0.163755730877703,0.503988317040579,-0.848044713969325));
#136940=DIRECTION('ref_axis',(-3.52263469559639E-16,0.85964918913047,0.510884792910619));
#136941=DIRECTION('center_axis',(-0.309016994374914,-0.951056516295164,
-1.50830667185725E-14));
#136942=DIRECTION('ref_axis',(-0.951056516295164,0.309016994374914,3.41480999208034E-15));
#136943=DIRECTION('center_axis',(0.309016994374914,0.951056516295165,6.64119215765945E-15));
#136944=DIRECTION('ref_axis',(0.951056516295164,-0.309016994374914,-3.41480999208033E-15));
#136945=DIRECTION('center_axis',(-0.309016994374938,-0.951056516295157,
-6.68470697498369E-15));
#136946=DIRECTION('ref_axis',(-0.951056516295156,0.309016994374938,3.41480999208031E-15));
#136947=DIRECTION('center_axis',(-0.309016994374914,-0.951056516295164,
1.80068240325357E-15));
#136948=DIRECTION('ref_axis',(-0.951056516295164,0.309016994374914,3.41480999208033E-15));
#136949=DIRECTION('center_axis',(-0.309016994374938,-0.951056516295157,
-6.68470697498369E-15));
#136950=DIRECTION('ref_axis',(-0.951056516295156,0.309016994374938,3.41480999208031E-15));
#136951=DIRECTION('center_axis',(0.267587483539828,0.823661100222926,0.499979330205141));
#136952=DIRECTION('ref_axis',(-0.153585232154563,-0.475806237439678,0.866036951219476));
#136953=DIRECTION('center_axis',(-0.154510091261949,-0.475533164204398,
-0.8660224254833));
#136954=DIRECTION('ref_axis',(-2.91289309623471E-16,0.876548714628845,-0.481313152617421));
#136955=DIRECTION('center_axis',(-0.1545100940345,-0.475533172737467,-0.866022420303128));
#136956=DIRECTION('ref_axis',(0.951056516295032,-0.309016994375322,2.70999320328836E-13));
#136957=DIRECTION('center_axis',(0.103956887954599,0.489078705158833,-0.866022508718425));
#136958=DIRECTION('ref_axis',(-0.978147600732856,0.207911690822227,2.63131599354494E-12));
#136959=DIRECTION('center_axis',(0.180084698745615,0.847087400906804,-0.500012436347994));
#136960=DIRECTION('ref_axis',(0.102990311575353,0.489291521303063,0.866017784403153));
#136961=DIRECTION('center_axis',(-0.103956889752271,-0.489078713616376,
0.866022503726309));
#136962=DIRECTION('ref_axis',(3.36406328257384E-16,-0.8707403454847,-0.491743073916843));
#136963=DIRECTION('center_axis',(-0.207911690817757,-0.978147600733806,
-6.83036818919254E-15));
#136964=DIRECTION('ref_axis',(-0.978147600733806,0.207911690817757,-2.9624920046404E-32));
#136965=DIRECTION('center_axis',(0.207911690817749,0.978147600733808,6.85964567039975E-15));
#136966=DIRECTION('ref_axis',(0.978147600733808,-0.207911690817749,-5.45082275808818E-31));
#136967=DIRECTION('center_axis',(0.207911690817754,0.978147600733807,6.83036818919254E-15));
#136968=DIRECTION('ref_axis',(0.978147600733807,-0.207911690817754,1.95361542122215E-29));
#136969=DIRECTION('center_axis',(0.207911690817749,0.978147600733808,6.85964567039975E-15));
#136970=DIRECTION('ref_axis',(0.978147600733808,-0.207911690817749,6.12351326823131E-31));
#136971=DIRECTION('center_axis',(-0.207911690817754,-0.978147600733807,
-6.83036818919254E-15));
#136972=DIRECTION('ref_axis',(-0.978147600733807,0.207911690817754,-1.95800148050649E-29));
#136973=DIRECTION('center_axis',(0.110177439185349,0.518344097776633,0.848045003637594));
#136974=DIRECTION('ref_axis',(6.77677416945363E-16,-0.853239582811881,0.521519140898018));
#136975=DIRECTION('center_axis',(-0.103956917928284,-0.489078846173993,
-0.866022425483294));
#136976=DIRECTION('ref_axis',(1.37107671501608E-16,0.870740269393781,-0.491743208652692));
#136977=DIRECTION('center_axis',(-0.110177412158605,-0.518344074628572,
-0.848045021297503));
#136978=DIRECTION('ref_axis',(-0.172101506927857,-0.830401496089509,0.529919264233209));
#136979=DIRECTION('center_axis',(0.110177427516376,0.518344042878429,0.848045038708628));
#136980=DIRECTION('ref_axis',(-1.64656692434778E-15,-0.853239616987284,
0.52151908498481));
#136981=DIRECTION('center_axis',(-0.103956910521484,-0.489078861909693,
-0.866022417485799));
#136982=DIRECTION('ref_axis',(-0.175605160694143,-0.848034685338789,0.499999999999924));
#136983=DIRECTION('center_axis',(-0.180092991631242,-0.847105178672024,
-0.499979330205107));
#136984=DIRECTION('ref_axis',(0.104894406044524,0.488852904975547,-0.866036951219482));
#136985=DIRECTION('center_axis',(0.978197989689811,-0.207674488001809,1.19112578788782E-14));
#136986=DIRECTION('ref_axis',(-0.207674488001809,-0.97819798968981,-6.82961998416062E-15));
#136987=DIRECTION('center_axis',(0.207911690817749,0.978147600733808,6.85964567039975E-15));
#136988=DIRECTION('ref_axis',(0.978147600733808,-0.207911690817749,-5.45082275808818E-31));
#136989=DIRECTION('center_axis',(-0.207911690817754,-0.978147600733807,
-6.83036818919254E-15));
#136990=DIRECTION('ref_axis',(-0.978147600733807,0.207911690817754,-1.95800148050649E-29));
#136991=DIRECTION('center_axis',(-1.70094388097117E-16,-7.12070239730339E-15,
1.));
#136992=DIRECTION('ref_axis',(-1.,1.20258066624967E-30,-1.69248182512655E-16));
#136993=DIRECTION('center_axis',(0.978097154258596,-0.208148881407602,-1.45349587027143E-15));
#136994=DIRECTION('ref_axis',(-0.208148881407602,-0.978097154258596,-6.82961998416085E-15));
#136995=DIRECTION('center_axis',(-0.110177535564893,-0.518344551206603,
0.8480447139693));
#136996=DIRECTION('ref_axis',(-2.8516928717058E-16,-0.853239300541027,-0.521519602711403));
#136997=DIRECTION('center_axis',(-0.11017742751637,-0.5183440428784,-0.848045038708647));
#136998=DIRECTION('ref_axis',(-5.45915083851553E-16,0.853239616987302,-0.52151908498478));
#136999=DIRECTION('center_axis',(-0.1101775670102,-0.518344577865721,0.848044693589271));
#137000=DIRECTION('ref_axis',(0.171882402212669,0.830446875606248,0.529919264233169));
#137001=DIRECTION('center_axis',(-0.110177549147491,-0.518344615107845,
0.848044673146735));
#137002=DIRECTION('ref_axis',(-1.38217757861089E-15,-0.853239260760969,
-0.521519667794107));
#137003=DIRECTION('center_axis',(0.110177412119122,0.518344074798825,0.84804502119857));
#137004=DIRECTION('ref_axis',(-0.180532167035008,-0.828609503964449,0.529919264233179));
#137005=DIRECTION('center_axis',(-0.110177439185351,-0.51834409777664,-0.84804500363759));
#137006=DIRECTION('ref_axis',(-9.47944080834145E-16,0.853239582811877,-0.521519140898025));
#137007=DIRECTION('center_axis',(0.978201246800566,-0.207659145615641,-1.45007606351424E-15));
#137008=DIRECTION('ref_axis',(-0.207659145615641,-0.978201246800566,-6.82961998416063E-15));
#137009=DIRECTION('center_axis',(-0.207911690817754,-0.978147600733807,
-3.9904525120933E-15));
#137010=DIRECTION('ref_axis',(-0.978147600733807,0.207911690817754,-1.14772778150505E-29));
#137011=DIRECTION('center_axis',(-1.70094388097117E-16,-7.12070239730339E-15,
1.));
#137012=DIRECTION('ref_axis',(-1.,1.28019500997425E-30,-1.72664287379267E-16));
#137013=DIRECTION('center_axis',(0.978093889466684,-0.208164222161096,-1.48136221419545E-14));
#137014=DIRECTION('ref_axis',(-0.208164222161096,-0.978093889466684,-6.8296199841606E-15));
#137015=DIRECTION('center_axis',(-0.207911690817749,-0.978147600733808,
-6.85964567039975E-15));
#137016=DIRECTION('ref_axis',(-0.978147600733808,0.207911690817749,-4.42564229104924E-29));
#137017=DIRECTION('center_axis',(-0.180025927304208,-0.847099893161378,
0.500012436349579));
#137018=DIRECTION('ref_axis',(-0.10492645952785,-0.488879980353024,-0.866017784402247));
#137019=DIRECTION('center_axis',(0.110177549147416,0.518344615107856,-0.848044673146738));
#137020=DIRECTION('ref_axis',(1.22718678990651E-15,0.853239260760965,0.521519667794113));
#137021=DIRECTION('center_axis',(0.103956896853785,0.489078698392239,-0.866022511471547));
#137022=DIRECTION('ref_axis',(0.184432991077372,0.846158656400951,0.499999999999992));
#137023=DIRECTION('center_axis',(-0.103956889752269,-0.489078713616277,
0.866022503726365));
#137024=DIRECTION('ref_axis',(1.91503290536032E-16,-0.870740345484756,-0.491743073916743));
#137025=DIRECTION('center_axis',(0.110177567037555,0.518344577661421,-0.84804469371059));
#137026=DIRECTION('ref_axis',(0.180750786626522,0.828561842307743,0.529919264233235));
#137027=DIRECTION('center_axis',(0.110177535564769,0.518344551206602,-0.848044713969317));
#137028=DIRECTION('ref_axis',(4.66838780246052E-16,0.853239300541032,0.521519602711394));
#137029=DIRECTION('center_axis',(-0.207911690817754,-0.978147600733807,
-6.83036818919254E-15));
#137030=DIRECTION('ref_axis',(-0.978147600733807,0.207911690817754,-1.95361542122215E-29));
#137031=DIRECTION('center_axis',(0.207911690817757,0.978147600733806,6.83036818919254E-15));
#137032=DIRECTION('ref_axis',(0.978147600733806,-0.207911690817757,2.9624920046404E-32));
#137033=DIRECTION('center_axis',(-0.207911690817749,-0.978147600733808,
-6.85964567039975E-15));
#137034=DIRECTION('ref_axis',(-0.978147600733808,0.207911690817749,-4.42564229104924E-29));
#137035=DIRECTION('center_axis',(-0.207911690817754,-0.978147600733807,
-1.15053683499437E-15));
#137036=DIRECTION('ref_axis',(-0.978147600733807,0.207911690817754,-3.31272147910634E-30));
#137037=DIRECTION('center_axis',(-0.207911690817749,-0.978147600733808,
-6.85964567039975E-15));
#137038=DIRECTION('ref_axis',(-0.978147600733808,0.207911690817749,-4.42564229104924E-29));
#137039=DIRECTION('center_axis',(0.180025582246976,0.847119506979154,0.499979330204792));
#137040=DIRECTION('ref_axis',(-0.103008581358723,-0.489253749386354,0.866036951219668));
#137041=DIRECTION('center_axis',(-0.103956917928285,-0.489078846173996,
-0.866022425483293));
#137042=DIRECTION('ref_axis',(7.50813757209353E-17,0.87074026939378,-0.491743208652695));
#137043=DIRECTION('center_axis',(-0.103956919794064,-0.489078854951829,
-0.866022420302118));
#137044=DIRECTION('ref_axis',(0.978147600734944,-0.207911690812404,-3.14708888126906E-12));
#137045=DIRECTION('center_axis',(0.052264755777796,0.497265934580814,-0.866022508719581));
#137046=DIRECTION('ref_axis',(-0.994521895368699,0.1045284632636,-2.36468762881567E-12));
#137047=DIRECTION('center_axis',(0.0905534316544205,0.86127094430961,-0.500012436348978));
#137048=DIRECTION('ref_axis',(0.0512812291455777,0.497376550146495,0.866017784402658));
#137049=DIRECTION('center_axis',(-0.052264756681742,-0.497265943181931,
0.866022503726308));
#137050=DIRECTION('ref_axis',(-5.67711925317034E-16,-0.867207748104371,
-0.497946504785149));
#137051=DIRECTION('center_axis',(-0.104528463267628,-0.994521895368276,
-6.94470927749848E-15));
#137052=DIRECTION('ref_axis',(-0.994521895368276,0.104528463267628,-1.09814391166396E-31));
#137053=DIRECTION('center_axis',(0.104528463267644,0.994521895368274,6.95942865237777E-15));
#137054=DIRECTION('ref_axis',(0.994521895368274,-0.104528463267644,2.54964018847027E-31));
#137055=DIRECTION('center_axis',(0.104528463267629,0.994521895368276,7.65859895914467E-15));
#137056=DIRECTION('ref_axis',(0.994521895368276,-0.104528463267629,-5.54203336120443E-30));
#137057=DIRECTION('center_axis',(0.104528463267644,0.994521895368274,6.95942865237777E-15));
#137058=DIRECTION('ref_axis',(0.994521895368274,-0.104528463267644,-3.92382721438483E-32));
#137059=DIRECTION('center_axis',(-0.10452846326763,-0.994521895368276,-6.94470927749848E-15));
#137060=DIRECTION('ref_axis',(-0.994521895368276,0.10452846326763,9.84955453724887E-30));
#137061=DIRECTION('center_axis',(0.0553921636609794,0.527021232978621,0.848045003637572));
#137062=DIRECTION('ref_axis',(8.12865720800958E-16,-0.849349030019372,0.527831625809927));
#137063=DIRECTION('center_axis',(-0.0522647708473857,-0.497266077958567,
-0.866022425483298));
#137064=DIRECTION('ref_axis',(1.39086404037747E-16,0.867207670398085,-0.497946640115912));
#137065=DIRECTION('center_axis',(-0.05539213919652,-0.527021207132817,-0.848045021297515));
#137066=DIRECTION('ref_axis',(-0.0843581245622004,-0.84384197585503,0.529919264233172));
#137067=DIRECTION('center_axis',(0.0553921577943494,0.527021177161365,0.848045038708638));
#137068=DIRECTION('ref_axis',(-7.11135774336482E-17,-0.849349064867508,
0.527831569734788));
#137069=DIRECTION('center_axis',(-0.052264761839755,-0.497266092833514,
-0.866022417485786));
#137070=DIRECTION('ref_axis',(-0.0859994148074141,-0.861744800189027,0.499999999999957));
#137071=DIRECTION('center_axis',(-0.0905598208270387,-0.861289491529733,
-0.499979330204988));
#137072=DIRECTION('ref_axis',(0.0532207405876983,0.4971393686821,-0.866036951219554));
#137073=DIRECTION('center_axis',(0.994547213842469,-0.104287292793425,1.2856524780366E-14));
#137074=DIRECTION('ref_axis',(-0.104287292793425,-0.994547213842469,-6.82961998416055E-15));
#137075=DIRECTION('center_axis',(0.104528463267644,0.994521895368274,6.95942865237777E-15));
#137076=DIRECTION('ref_axis',(0.994521895368274,-0.104528463267644,2.54964018847027E-31));
#137077=DIRECTION('center_axis',(-0.104528463267628,-0.994521895368276,
-6.94470927749848E-15));
#137078=DIRECTION('ref_axis',(-0.994521895368276,0.104528463267628,-1.09814391166396E-31));
#137079=DIRECTION('center_axis',(-1.55536281769216E-16,-7.12300817482632E-15,
1.));
#137080=DIRECTION('ref_axis',(-1.,1.20258066624967E-30,-1.55144167303267E-16));
#137081=DIRECTION('center_axis',(0.994496518411992,-0.104769627595152,-7.31602399252034E-16));
#137082=DIRECTION('ref_axis',(-0.104769627595152,-0.994496518411992,-6.82961998416046E-15));
#137083=DIRECTION('center_axis',(-0.055392212116204,-0.527021693999024,
0.848044713969301));
#137084=DIRECTION('ref_axis',(-3.41086766092002E-17,-0.849348742192385,
-0.527832088960318));
#137085=DIRECTION('center_axis',(-0.0553921577943474,-0.527021177161346,
-0.84804503870865));
#137086=DIRECTION('ref_axis',(3.58151228089054E-16,0.84934906486752,-0.527831569734768));
#137087=DIRECTION('center_axis',(-0.0553922405964155,-0.527021723799658,
0.848044693589286));
#137088=DIRECTION('ref_axis',(0.0841354767083805,0.843864204095404,0.529919264233227));
#137089=DIRECTION('center_axis',(-0.0553922189449436,-0.527021758969977,
0.848044673146732));
#137090=DIRECTION('ref_axis',(-5.11211380535554E-17,-0.849348701629307,
-0.527832154231447));
#137091=DIRECTION('center_axis',(0.0553921391546639,0.5270212072964,0.848045021198589));
#137092=DIRECTION('ref_axis',(-0.0929299148097542,-0.842941044396323,0.52991926423323));
#137093=DIRECTION('center_axis',(-0.0553921636609763,-0.527021232978591,
-0.848045003637591));
#137094=DIRECTION('ref_axis',(-1.63069853500586E-16,0.849349030019391,-0.527831625809898));
#137095=DIRECTION('center_axis',(0.994548849394384,-0.104271693993661,3.67176988899929E-16));
#137096=DIRECTION('ref_axis',(-0.104271693993661,-0.994548849394384,-6.82961998416081E-15));
#137097=DIRECTION('center_axis',(-0.104528463267629,-0.994521895368276,
-6.94470927749848E-15));
#137098=DIRECTION('ref_axis',(-0.994521895368276,0.104528463267629,4.91917387961755E-30));
#137099=DIRECTION('center_axis',(-1.55536281769216E-16,-7.12300817482632E-15,
1.));
#137100=DIRECTION('ref_axis',(-1.,1.28019500997425E-30,-1.576500015202E-16));
#137101=DIRECTION('center_axis',(0.99449487505034,-0.104785225574074,-7.31711319356696E-16));
#137102=DIRECTION('ref_axis',(-0.104785225574074,-0.994494875050339,-6.82961998416066E-15));
#137103=DIRECTION('center_axis',(-0.104528463267644,-0.994521895368274,
-6.95942865237777E-15));
#137104=DIRECTION('ref_axis',(-0.994521895368274,0.104528463267644,9.55177901418214E-30));
#137105=DIRECTION('center_axis',(-0.0904936763714717,-0.861277224842458,
0.500012436349786));
#137106=DIRECTION('ref_axis',(-0.053249788305639,-0.497169646242195,-0.866017784402154));
#137107=DIRECTION('center_axis',(0.0553922189448982,0.527021758969989,-0.848044673146727));
#137108=DIRECTION('ref_axis',(-1.85765759131825E-16,0.8493487016293,0.527832154231458));
#137109=DIRECTION('center_axis',(0.052264765337821,0.497265928783258,-0.866022511471559));
#137110=DIRECTION('ref_axis',(0.0949749838233155,0.860801807879023,0.499999999999967));
#137111=DIRECTION('center_axis',(-0.0522647566817781,-0.497265943181826,
0.866022503726366));
#137112=DIRECTION('ref_axis',(7.61153916252116E-16,-0.867207748104431,-0.497946504785044));
#137113=DIRECTION('center_axis',(0.0553922406558896,0.527021723598192,-0.848044693710603));
#137114=DIRECTION('ref_axis',(0.0931523188145091,0.842916495801343,0.529919264233209));
#137115=DIRECTION('center_axis',(0.0553922121161434,0.527021693999006,-0.848044713969316));
#137116=DIRECTION('ref_axis',(3.67189309331813E-16,0.849348742192398,0.527832088960298));
#137117=DIRECTION('center_axis',(-0.104528463267629,-0.994521895368276,
-6.23081959585225E-15));
#137118=DIRECTION('ref_axis',(-0.994521895368276,0.104528463267629,4.46057211924954E-30));
#137119=DIRECTION('center_axis',(0.104528463267629,0.994521895368276,6.94470927749848E-15));
#137120=DIRECTION('ref_axis',(0.994521895368276,-0.104528463267629,-4.99922698313062E-30));
#137121=DIRECTION('center_axis',(-0.104528463267644,-0.994521895368274,
-6.95942865237777E-15));
#137122=DIRECTION('ref_axis',(-0.994521895368274,0.104528463267644,9.55177901418214E-30));
#137123=DIRECTION('center_axis',(-0.104528463267629,-0.994521895368276,
-6.94470927749848E-15));
#137124=DIRECTION('ref_axis',(-0.994521895368276,0.104528463267629,4.99922698313062E-30));
#137125=DIRECTION('center_axis',(-0.104528463267644,-0.994521895368274,
-6.95942865237777E-15));
#137126=DIRECTION('ref_axis',(-0.994521895368274,0.104528463267644,9.55177901418214E-30));
#137127=DIRECTION('center_axis',(0.0904912830026074,0.861296695145313,0.499979330205064));
#137128=DIRECTION('ref_axis',(-0.0513033469953135,-0.497340894869405,0.866036951219507));
#137129=DIRECTION('center_axis',(-0.0522647708473827,-0.497266077958539,
-0.866022425483315));
#137130=DIRECTION('ref_axis',(6.35438415383309E-16,0.867207670398102,-0.497946640115884));
#137131=DIRECTION('center_axis',(-0.0522647717855476,-0.497266086884524,
-0.866022420301436));
#137132=DIRECTION('ref_axis',(0.994521895367887,-0.104528463271327,2.15051073550011E-12));
#137133=DIRECTION('center_axis',(-5.08733525851855E-15,0.500005014362956,
-0.86602250872128));
#137134=DIRECTION('ref_axis',(-1.,-2.37780049919996E-12,-1.38122234879998E-12));
#137135=DIRECTION('center_axis',(3.00422159424583E-5,0.866018223014576,
-0.500012436349478));
#137136=DIRECTION('ref_axis',(-0.000989701280057339,0.500012217440974,0.866017784402339));
#137137=DIRECTION('center_axis',(-2.73187543788774E-14,-0.500005023014378,
0.866022503726313));
#137138=DIRECTION('ref_axis',(1.77159806316853E-29,-0.866022503726313,-0.500005023014378));
#137139=DIRECTION('center_axis',(0.,-1.,-6.98296267768627E-15));
#137140=DIRECTION('ref_axis',(0.,6.98296267768627E-15,-1.));
#137141=DIRECTION('center_axis',(-1.04744440165294E-14,1.,6.98296267768627E-15));
#137142=DIRECTION('ref_axis',(1.,1.04744440165294E-14,-1.12103877145985E-44));
#137143=DIRECTION('center_axis',(0.,1.,6.98296267768627E-15));
#137144=DIRECTION('ref_axis',(0.,-6.98296267768627E-15,1.));
#137145=DIRECTION('center_axis',(-1.04744440165294E-14,1.,6.98296267768627E-15));
#137146=DIRECTION('ref_axis',(1.,1.04744440165294E-14,-1.12103877145985E-44));
#137147=DIRECTION('center_axis',(0.,-1.,-6.98296267768627E-15));
#137148=DIRECTION('ref_axis',(0.,6.98296267768627E-15,-1.));
#137149=DIRECTION('center_axis',(0.,0.529924213265784,0.848045003637567));
#137150=DIRECTION('ref_axis',(0.,-0.848045003637567,0.529924213265784));
#137151=DIRECTION('center_axis',(0.,-0.500005158533416,-0.866022425483298));
#137152=DIRECTION('ref_axis',(0.,0.866022425483298,-0.500005158533416));
#137153=DIRECTION('center_axis',(2.16260202548866E-8,-0.529924185004347,
-0.848045021297501));
#137154=DIRECTION('ref_axis',(0.00430950302111146,-0.848037146343372,0.529919264233243));
#137155=DIRECTION('center_axis',(0.,0.529924157141045,0.848045038708648));
#137156=DIRECTION('ref_axis',(0.,-0.848045038708648,0.529924157141045));
#137157=DIRECTION('center_axis',(1.05155814435434E-8,-0.500005172385354,
-0.866022417485767));
#137158=DIRECTION('ref_axis',(0.00454855868473161,-0.866013458679421,0.499999999999998));
#137159=DIRECTION('center_axis',(-3.44576747652515E-5,-0.86603733648169,
-0.499979330205127));
#137160=DIRECTION('ref_axis',(0.000963977567144606,0.499979069431645,-0.866036951219471));
#137161=DIRECTION('center_axis',(-1.04744440165294E-14,1.,6.98296267768627E-15));
#137162=DIRECTION('ref_axis',(1.,1.04744440165294E-14,-1.12103877145985E-44));
#137163=DIRECTION('center_axis',(0.,-1.,-6.98296267768627E-15));
#137164=DIRECTION('ref_axis',(0.,6.98296267768627E-15,-1.));
#137165=DIRECTION('center_axis',(-2.89534733035821E-14,-0.529924676825572,
0.848044713969324));
#137166=DIRECTION('ref_axis',(6.94515430910295E-29,-0.848044713969324,-0.529924676825572));
#137167=DIRECTION('center_axis',(0.,-0.529924157141035,-0.848045038708655));
#137168=DIRECTION('ref_axis',(0.,0.848045038708655,-0.529924157141035));
#137169=DIRECTION('center_axis',(-2.52127146216552E-8,-0.529924709439994,
0.848044693589281));
#137170=DIRECTION('ref_axis',(-0.00453325470002202,0.848035979777022,0.529919264233195));
#137171=DIRECTION('center_axis',(-4.63345827774717E-14,-0.529924742154438,
0.848044673146735));
#137172=DIRECTION('ref_axis',(-3.13786732617605E-28,-0.848044673146735,
-0.529924742154438));
#137173=DIRECTION('center_axis',(-2.16960312490591E-8,0.529924185162669,
0.848045021198569));
#137174=DIRECTION('ref_axis',(-0.00430950303215927,-0.848037146343347,0.529919264233193));
#137175=DIRECTION('center_axis',(0.,-0.529924213265784,-0.848045003637567));
#137176=DIRECTION('ref_axis',(0.,0.848045003637567,-0.529924213265784));
#137177=DIRECTION('center_axis',(0.,-1.,-6.98296267768627E-15));
#137178=DIRECTION('ref_axis',(0.,6.98296267768627E-15,-1.));
#137179=DIRECTION('center_axis',(1.04744440165294E-14,-1.,-6.98296267768627E-15));
#137180=DIRECTION('ref_axis',(-1.,-1.04744440165294E-14,-1.34524652575182E-42));
#137181=DIRECTION('center_axis',(3.00422162114182E-5,-0.86601822301478,
0.500012436349125));
#137182=DIRECTION('ref_axis',(-0.000989701260860521,-0.50001221744063,-0.86601778440256));
#137183=DIRECTION('center_axis',(0.,0.529924742154438,-0.848044673146735));
#137184=DIRECTION('ref_axis',(0.,0.848044673146735,0.529924742154438));
#137185=DIRECTION('center_axis',(1.01126011638448E-8,0.500005009599381,
-0.866022511471569));
#137186=DIRECTION('ref_axis',(0.00447641076763253,0.866013834616223,0.499999999999945));
#137187=DIRECTION('center_axis',(0.,-0.500005023014361,0.866022503726323));
#137188=DIRECTION('ref_axis',(0.,-0.866022503726323,-0.500005023014361));
#137189=DIRECTION('center_axis',(2.52898507296124E-8,0.529924709245839,
-0.848044693710604));
#137190=DIRECTION('ref_axis',(0.0045332546887403,0.848035979777057,0.529919264233236));
#137191=DIRECTION('center_axis',(-2.89534733035821E-14,0.529924676825572,
-0.848044713969324));
#137192=DIRECTION('ref_axis',(6.64353622666922E-29,0.848044713969324,0.529924676825572));
#137193=DIRECTION('center_axis',(0.,-1.,-6.98296267768627E-15));
#137194=DIRECTION('ref_axis',(0.,6.98296267768627E-15,-1.));
#137195=DIRECTION('center_axis',(0.,1.,6.98296267768627E-15));
#137196=DIRECTION('ref_axis',(0.,-6.98296267768627E-15,1.));
#137197=DIRECTION('center_axis',(1.04744440165294E-14,-1.,-6.98296267768627E-15));
#137198=DIRECTION('ref_axis',(-1.,-1.04744440165294E-14,-1.34524652575182E-42));
#137199=DIRECTION('center_axis',(0.,-1.,-6.98296267768627E-15));
#137200=DIRECTION('ref_axis',(0.,6.98296267768627E-15,-1.));
#137201=DIRECTION('center_axis',(1.04744440165294E-14,-1.,-6.98296267768627E-15));
#137202=DIRECTION('ref_axis',(-1.,-1.04744440165294E-14,-1.34524652575182E-42));
#137203=DIRECTION('center_axis',(-3.44576744698565E-5,0.866037336481585,
0.49997933020531));
#137204=DIRECTION('ref_axis',(0.000963977573258117,-0.499979069431825,0.86603695121936));
#137205=DIRECTION('center_axis',(0.,-0.500005158533416,-0.866022425483298));
#137206=DIRECTION('ref_axis',(0.,0.866022425483298,-0.500005158533416));
#137207=DIRECTION('center_axis',(5.43770948728685E-15,-0.500005167508441,
-0.866022420301493));
#137208=DIRECTION('ref_axis',(1.,-1.39870616943407E-13,6.99353084717037E-14));
#137209=DIRECTION('center_axis',(-0.0522647557774501,0.49726593457756,-0.866022508721471));
#137210=DIRECTION('ref_axis',(-0.99452189536814,-0.104528463268923,-7.21207871993735E-13));
#137211=DIRECTION('center_axis',(-0.090493676372131,0.86127722484266,-0.50001243634932));
#137212=DIRECTION('ref_axis',(-0.0532497883196993,0.497169646240241,0.866017784402411));
#137213=DIRECTION('center_axis',(0.0522647566817887,-0.49726594318193,0.866022503726306));
#137214=DIRECTION('ref_axis',(5.67333325818785E-16,-0.867207748104371,-0.497946504785149));
#137215=DIRECTION('center_axis',(0.104528463267683,-0.99452189536827,-6.94470927749844E-15));
#137216=DIRECTION('ref_axis',(-0.99452189536827,-0.104528463267683,5.29715191372443E-32));
#137217=DIRECTION('center_axis',(-0.104528463267664,0.994521895368272,6.92998990261914E-15));
#137218=DIRECTION('ref_axis',(0.994521895368272,0.104528463267664,9.86230019548369E-32));
#137219=DIRECTION('center_axis',(-0.104528463267683,0.99452189536827,6.94470927749844E-15));
#137220=DIRECTION('ref_axis',(0.99452189536827,0.104528463267683,-5.29715191372443E-32));
#137221=DIRECTION('center_axis',(-0.104528463267664,0.994521895368272,6.92998990261914E-15));
#137222=DIRECTION('ref_axis',(0.994521895368272,0.104528463267664,-1.95579289036037E-31));
#137223=DIRECTION('center_axis',(0.104528463267682,-0.994521895368271,-6.94470927749844E-15));
#137224=DIRECTION('ref_axis',(-0.994521895368271,-0.104528463267682,9.97523142827348E-30));
#137225=DIRECTION('center_axis',(-0.055392163661009,0.527021232978627,0.848045003637566));
#137226=DIRECTION('ref_axis',(6.51171922772032E-16,-0.849349030019368,0.527831625809934));
#137227=DIRECTION('center_axis',(0.052264770847414,-0.497266077958576,-0.866022425483291));
#137228=DIRECTION('ref_axis',(-4.78888614370566E-17,0.86720767039808,-0.497946640115922));
#137229=DIRECTION('center_axis',(0.0553921822204516,-0.527021202610803,
-0.848045021297525));
#137230=DIRECTION('ref_axis',(0.092929914822725,-0.842941044394914,0.529919264233196));
#137231=DIRECTION('center_axis',(-0.0553921577943759,0.527021177161342,
0.848045038708651));
#137232=DIRECTION('ref_axis',(4.28784163588954E-16,-0.849349064867522,0.527831569734765));
#137233=DIRECTION('center_axis',(0.0522647827543777,-0.497266090635353,
-0.866022417485755));
#137234=DIRECTION('ref_axis',(0.0950466972129526,-0.860793892490479,0.5));
#137235=DIRECTION('center_axis',(0.0904912830030132,-0.861296695145195,
-0.499979330205193));
#137236=DIRECTION('ref_axis',(-0.0513033469930341,0.497340894869774,-0.86603695121943));
#137237=DIRECTION('center_axis',(0.994496518411991,0.104769627595163,-6.0604308970725E-15));
#137238=DIRECTION('ref_axis',(0.104769627595163,-0.994496518411991,-6.82961998416045E-15));
#137239=DIRECTION('center_axis',(-0.104528463267664,0.994521895368272,6.92998990261914E-15));
#137240=DIRECTION('ref_axis',(0.994521895368272,0.104528463267664,9.86230019548369E-32));
#137241=DIRECTION('center_axis',(0.104528463267628,-0.994521895368276,-6.94470927749848E-15));
#137242=DIRECTION('ref_axis',(-0.994521895368276,-0.104528463267628,1.09814391166396E-31));
#137243=DIRECTION('center_axis',(-1.26097532010602E-16,-7.12300817482632E-15,
1.));
#137244=DIRECTION('ref_axis',(0.,-1.,-7.12252768074091E-15));
#137245=DIRECTION('center_axis',(0.994547213842467,0.104287292793444,7.28234273333559E-16));
#137246=DIRECTION('ref_axis',(0.104287292793444,-0.994547213842467,-6.82961998416053E-15));
#137247=DIRECTION('center_axis',(0.0553922121162013,-0.527021693998998,
0.848044713969317));
#137248=DIRECTION('ref_axis',(4.11774601795882E-16,-0.849348742192401,-0.527832088960292));
#137249=DIRECTION('center_axis',(0.0553921577943754,-0.527021177161337,
-0.848045038708654));
#137250=DIRECTION('ref_axis',(-5.92818387691785E-16,0.849349064867525,-0.52783156973476));
#137251=DIRECTION('center_axis',(0.055392190456375,-0.527021729069563,0.848044693589302));
#137252=DIRECTION('ref_axis',(-0.0931523188057552,0.842916495802302,0.529919264233221));
#137253=DIRECTION('center_axis',(0.0553922189449272,-0.527021758969985,
0.848044673146728));
#137254=DIRECTION('ref_axis',(-1.43295946606909E-16,-0.849348701629302,
-0.527832154231455));
#137255=DIRECTION('center_axis',(-0.0553921822983099,0.527021202761856,
0.848045021198567));
#137256=DIRECTION('ref_axis',(0.0843581245724762,-0.843841975853982,0.529919264233205));
#137257=DIRECTION('center_axis',(0.0553921636610064,-0.527021232978603,
-0.848045003637582));
#137258=DIRECTION('ref_axis',(4.73641288854564E-16,0.849349030019383,-0.52783162580991));
#137259=DIRECTION('center_axis',(0.994494875050337,0.104785225574097,1.79858722714094E-15));
#137260=DIRECTION('ref_axis',(0.104785225574097,-0.994494875050337,-6.82961998416065E-15));
#137261=DIRECTION('center_axis',(0.104528463267683,-0.99452189536827,-7.658598959145E-15));
#137262=DIRECTION('ref_axis',(-0.99452189536827,-0.104528463267683,5.02333238162146E-32));
#137263=DIRECTION('center_axis',(-1.26097532010602E-16,-7.12300817482632E-15,
1.));
#137264=DIRECTION('ref_axis',(0.,-1.,-7.12427864012715E-15));
#137265=DIRECTION('center_axis',(0.994548849394382,0.104271693993677,-3.67176988898936E-16));
#137266=DIRECTION('ref_axis',(0.104271693993677,-0.994548849394382,-6.82961998416079E-15));
#137267=DIRECTION('center_axis',(0.104528463267664,-0.994521895368272,-6.92998990261914E-15));
#137268=DIRECTION('ref_axis',(-0.994521895368272,-0.104528463267664,-5.68846653078145E-30));
#137269=DIRECTION('center_axis',(0.090553431653363,-0.861270944310248,0.50001243634807));
#137270=DIRECTION('ref_axis',(0.0512812291155024,-0.497376550148729,-0.866017784403157));
#137271=DIRECTION('center_axis',(-0.0553922189449268,0.527021758969978,
-0.848044673146732));
#137272=DIRECTION('ref_axis',(-1.82739123987317E-17,0.849348701629307,0.527832154231448));
#137273=DIRECTION('center_axis',(-0.0522647452170547,0.497265930897975,
-0.866022511471594));
#137274=DIRECTION('ref_axis',(-0.0860712067688574,0.861737632557287,0.499999999999914));
#137275=DIRECTION('center_axis',(0.0522647566818046,-0.497265943181818,
0.866022503726369));
#137276=DIRECTION('ref_axis',(-6.46601314095184E-16,-0.867207748104435,
-0.497946504785037));
#137277=DIRECTION('center_axis',(-0.0553921903530692,0.527021728885246,
-0.848044693710594));
#137278=DIRECTION('ref_axis',(-0.0841354767237599,0.843864204093855,0.529919264233251));
#137279=DIRECTION('center_axis',(-0.0553922121162459,0.527021693998979,
-0.848044713969325));
#137280=DIRECTION('ref_axis',(-7.69598135871256E-16,0.849348742192412,0.527832088960275));
#137281=DIRECTION('center_axis',(0.104528463267683,-0.99452189536827,4.66790539311939E-14));
#137282=DIRECTION('ref_axis',(-0.99452189536827,-0.104528463267683,4.68802147627136E-31));
#137283=DIRECTION('center_axis',(-0.104528463267684,0.99452189536827,6.94470927749844E-15));
#137284=DIRECTION('ref_axis',(0.99452189536827,0.104528463267684,4.95746224200719E-30));
#137285=DIRECTION('center_axis',(0.104528463267664,-0.994521895368272,-6.92998990261914E-15));
#137286=DIRECTION('ref_axis',(-0.994521895368272,-0.104528463267664,-5.68846653078145E-30));
#137287=DIRECTION('center_axis',(0.104528463267683,-0.99452189536827,-1.62252751389037E-14));
#137288=DIRECTION('ref_axis',(-0.99452189536827,-0.104528463267683,2.5477722298887E-32));
#137289=DIRECTION('center_axis',(0.104528463267664,-0.994521895368272,-6.92998990261914E-15));
#137290=DIRECTION('ref_axis',(-0.994521895368272,-0.104528463267664,-5.68846653078145E-30));
#137291=DIRECTION('center_axis',(-0.0905598208268657,0.861289491529602,
0.499979330205246));
#137292=DIRECTION('ref_axis',(0.0532207405971731,-0.497139368681358,0.866036951219397));
#137293=DIRECTION('center_axis',(0.0522647708474102,-0.49726607795854,-0.866022425483312));
#137294=DIRECTION('ref_axis',(-4.9818014384587E-16,0.8672076703981,-0.497946640115886));
#137295=DIRECTION('center_axis',(0.0522647717853422,-0.497266086882506,
-0.866022420302607));
#137296=DIRECTION('ref_axis',(0.994521895368341,0.104528463267008,3.93386110152788E-13));
#137297=DIRECTION('center_axis',(-0.103956887952778,0.489078705150286,-0.86602250872347));
#137298=DIRECTION('ref_axis',(-0.97814760073492,-0.207911690812515,3.12086315513693E-12));
#137299=DIRECTION('center_axis',(-0.180025927304753,0.847099893162251,-0.500012436347904));
#137300=DIRECTION('ref_axis',(-0.104926459563228,0.488879980343774,0.866017784403182));
#137301=DIRECTION('center_axis',(0.103956889752339,-0.48907871361637,0.866022503726305));
#137302=DIRECTION('ref_axis',(2.04314265460328E-17,-0.870740345484702,-0.49174307391684));
#137303=DIRECTION('center_axis',(0.207911690817757,-0.978147600733806,-6.3113295077734E-14));
#137304=DIRECTION('ref_axis',(-0.978147600733806,-0.207911690817757,-1.09041577388121E-30));
#137305=DIRECTION('center_axis',(-0.20791169081777,0.978147600733803,6.80109070798531E-15));
#137306=DIRECTION('ref_axis',(0.978147600733803,0.20791169081777,2.06817330173051E-31));
#137307=DIRECTION('center_axis',(-0.207911690817757,0.978147600733806,9.67028386629166E-15));
#137308=DIRECTION('ref_axis',(0.978147600733806,0.207911690817757,2.88043565065189E-31));
#137309=DIRECTION('center_axis',(-0.20791169081777,0.978147600733803,6.80109070798531E-15));
#137310=DIRECTION('ref_axis',(0.978147600733803,0.20791169081777,-3.71899471142921E-31));
#137311=DIRECTION('center_axis',(0.207911690817754,-0.978147600733807,-6.83036818919254E-15));
#137312=DIRECTION('ref_axis',(-0.978147600733807,-0.207911690817754,1.95800148050649E-29));
#137313=DIRECTION('center_axis',(-0.110177439185351,0.518344097776635,0.848045003637592));
#137314=DIRECTION('ref_axis',(-7.54079398017999E-16,-0.853239582811879,
0.521519140898021));
#137315=DIRECTION('center_axis',(0.103956917928287,-0.489078846173993,-0.866022425483294));
#137316=DIRECTION('ref_axis',(-1.22527346747099E-16,0.870740269393781,-0.491743208652692));
#137317=DIRECTION('center_axis',(0.110177454462975,-0.518344065636496,-0.848045021297506));
#137318=DIRECTION('ref_axis',(0.180532167026837,-0.828609503966227,0.529919264233183));
#137319=DIRECTION('center_axis',(-0.110177427516368,0.518344042878384,0.848045038708657));
#137320=DIRECTION('ref_axis',(1.77194910663906E-17,-0.853239616987312,0.521519084984763));
#137321=DIRECTION('center_axis',(0.103956931096973,-0.489078857536295,-0.866022417485767));
#137322=DIRECTION('ref_axis',(0.184503484229001,-0.846143288283582,0.500000000000006));
#137323=DIRECTION('center_axis',(0.180025582247408,-0.847119506978821,-0.4999793302052));
#137324=DIRECTION('ref_axis',(-0.1030085813648,0.489253749385483,-0.866036951219438));
#137325=DIRECTION('center_axis',(0.978097154258593,0.208148881407615,1.45349587027152E-15));
#137326=DIRECTION('ref_axis',(0.208148881407615,-0.978097154258593,-6.82961998416083E-15));
#137327=DIRECTION('center_axis',(-0.20791169081777,0.978147600733803,6.80109070798531E-15));
#137328=DIRECTION('ref_axis',(0.978147600733803,0.20791169081777,2.06817330173051E-31));
#137329=DIRECTION('center_axis',(0.207911690817809,-0.978147600733795,-6.83036818919246E-15));
#137330=DIRECTION('ref_axis',(-0.978147600733795,-0.207911690817809,-7.01020655912049E-32));
#137331=DIRECTION('center_axis',(-1.11539425682701E-16,-7.12070239730339E-15,
1.));
#137332=DIRECTION('ref_axis',(0.,-1.,-7.12252768074091E-15));
#137333=DIRECTION('center_axis',(0.978197989689803,0.207674488001846,1.45018319882449E-15));
#137334=DIRECTION('ref_axis',(0.207674488001846,-0.978197989689803,-6.82961998416081E-15));
#137335=DIRECTION('center_axis',(0.110177535564859,-0.51834455120658,0.848044713969319));
#137336=DIRECTION('ref_axis',(1.07836950919692E-15,-0.853239300541042,-0.521519602711377));
#137337=DIRECTION('center_axis',(0.110177427516366,-0.518344042878376,-0.848045038708663));
#137338=DIRECTION('ref_axis',(-4.28442985045855E-16,0.853239616987318,-0.521519084984755));
#137339=DIRECTION('center_axis',(0.110177517683837,-0.51834458835035,0.848044693589279));
#137340=DIRECTION('ref_axis',(-0.180750786636256,0.828561842305646,0.529919264233193));
#137341=DIRECTION('center_axis',(0.110177549147491,-0.518344615107838,0.848044673146739));
#137342=DIRECTION('ref_axis',(-1.48578503604637E-15,-0.853239260760973,
-0.5215196677941));
#137343=DIRECTION('center_axis',(-0.110177454559654,0.518344065777824,0.848045021198563));
#137344=DIRECTION('ref_axis',(0.172101506923684,-0.83040149609036,0.529919264233232));
#137345=DIRECTION('center_axis',(0.110177439185354,-0.518344097776646,-0.848045003637586));
#137346=DIRECTION('ref_axis',(1.16028044961569E-15,0.853239582811873,-0.521519140898032));
#137347=DIRECTION('center_axis',(0.978093889466681,0.20816422216111,1.68001810364593E-14));
#137348=DIRECTION('ref_axis',(0.20816422216111,-0.978093889466681,-6.82961998416056E-15));
#137349=DIRECTION('center_axis',(0.207911690817757,-0.978147600733806,-6.02733794006349E-14));
#137350=DIRECTION('ref_axis',(-0.978147600733806,-0.207911690817757,-7.42579907703451E-31));
#137351=DIRECTION('center_axis',(-1.11539425682701E-16,-7.12070239730339E-15,
1.));
#137352=DIRECTION('ref_axis',(0.,-1.,-7.11677149719761E-15));
#137353=DIRECTION('center_axis',(0.978201246800563,0.207659145615657,-5.65545097522343E-16));
#137354=DIRECTION('ref_axis',(0.207659145615657,-0.978201246800563,-6.8296199841606E-15));
#137355=DIRECTION('center_axis',(0.20791169081777,-0.978147600733803,-6.80109070798531E-15));
#137356=DIRECTION('ref_axis',(-0.978147600733803,-0.20791169081777,-3.10040133675291E-30));
#137357=DIRECTION('center_axis',(0.18008469874673,-0.847087400907193,0.500012436346933));
#137358=DIRECTION('ref_axis',(0.102990311599812,-0.489291521296793,-0.866017784403787));
#137359=DIRECTION('center_axis',(-0.110177549147563,0.518344615107829,-0.848044673146735));
#137360=DIRECTION('ref_axis',(1.43134731509193E-15,0.853239260760976,0.521519667794094));
#137361=DIRECTION('center_axis',(-0.103956877074907,0.489078702596384,-0.866022511471538));
#137362=DIRECTION('ref_axis',(-0.175675810178005,0.84802005266285,0.499999999999998));
#137363=DIRECTION('center_axis',(0.103956889752269,-0.489078713616267,0.866022503726371));
#137364=DIRECTION('ref_axis',(1.23480565415998E-16,-0.870740345484762,-0.491743073916733));
#137365=DIRECTION('center_axis',(-0.110177517565485,0.518344588177,-0.848044693710611));
#137366=DIRECTION('ref_axis',(-0.171882402212725,0.830446875606225,0.529919264233187));
#137367=DIRECTION('center_axis',(-0.110177535564811,0.518344551206578,-0.848044713969326));
#137368=DIRECTION('ref_axis',(-1.34557089476936E-15,0.853239300541045,0.521519602711372));
#137369=DIRECTION('center_axis',(0.207911690817757,-0.978147600733806,-6.02733794006349E-14));
#137370=DIRECTION('ref_axis',(-0.978147600733806,-0.207911690817757,-7.42579907703451E-31));
#137371=DIRECTION('center_axis',(-0.207911690817757,0.978147600733806,6.83036818919254E-15));
#137372=DIRECTION('ref_axis',(0.978147600733806,0.207911690817757,-2.9624920046404E-32));
#137373=DIRECTION('center_axis',(0.20791169081777,-0.978147600733803,-6.80109070798531E-15));
#137374=DIRECTION('ref_axis',(-0.978147600733803,-0.20791169081777,-3.10040133675291E-30));
#137375=DIRECTION('center_axis',(0.207911690817757,-0.978147600733806,6.64920527619437E-14));
#137376=DIRECTION('ref_axis',(-0.978147600733806,-0.207911690817757,-8.88628001461481E-31));
#137377=DIRECTION('center_axis',(0.20791169081777,-0.978147600733803,-6.80109070798531E-15));
#137378=DIRECTION('ref_axis',(-0.978147600733803,-0.20791169081777,-3.10040133675291E-30));
#137379=DIRECTION('center_axis',(-0.180092991631637,0.847105178672107,0.499979330204825));
#137380=DIRECTION('ref_axis',(0.104894406035295,-0.488852904977225,0.866036951219652));
#137381=DIRECTION('center_axis',(0.103956917928286,-0.489078846173992,-0.866022425483294));
#137382=DIRECTION('ref_axis',(-1.63962562710755E-16,0.870740269393781,-0.491743208652692));
#137383=DIRECTION('center_axis',(0.103956919794063,-0.489078854951801,-0.866022420302134));
#137384=DIRECTION('ref_axis',(0.978147600733311,0.207911690820085,-1.38559329909464E-12));
#137385=DIRECTION('center_axis',(-0.154510046710727,0.475533027089821,-0.866022508721477));
#137386=DIRECTION('ref_axis',(-0.951056516296016,-0.309016994372293,1.60414114558784E-12));
#137387=DIRECTION('center_axis',(-0.267585776505592,0.823641557783929,-0.5000124363485));
#137388=DIRECTION('ref_axis',(-0.15545353447606,0.475234043095452,0.866017784402867));
#137389=DIRECTION('center_axis',(0.154510049384266,-0.475533035318153,0.866022503726304));
#137390=DIRECTION('ref_axis',(2.11507007819763E-15,-0.876548788012429,-0.481313018974079));
#137391=DIRECTION('center_axis',(0.309016994374964,-0.951056516295148,-6.64119215765934E-15));
#137392=DIRECTION('ref_axis',(-0.951056516295148,-0.309016994374964,-3.41480999208031E-15));
#137393=DIRECTION('center_axis',(-0.309016994374957,0.95105651629515,6.59767734033506E-15));
#137394=DIRECTION('ref_axis',(0.95105651629515,0.309016994374957,3.41480999208033E-15));
#137395=DIRECTION('center_axis',(-0.309016994374964,0.951056516295148,6.64119215765934E-15));
#137396=DIRECTION('ref_axis',(0.951056516295148,0.309016994374964,3.41480999208031E-15));
#137397=DIRECTION('center_axis',(-0.309016994374957,0.95105651629515,6.59767734033506E-15));
#137398=DIRECTION('ref_axis',(0.95105651629515,0.309016994374957,3.41480999208033E-15));
#137399=DIRECTION('center_axis',(0.309016994374914,-0.951056516295165,-6.64119215765945E-15));
#137400=DIRECTION('ref_axis',(-0.951056516295164,-0.309016994374914,-3.41480999208033E-15));
#137401=DIRECTION('center_axis',(-0.163755587629897,0.50398787616896,0.848045003637595));
#137402=DIRECTION('ref_axis',(1.40487114752366E-15,-0.859649462041503,0.510884333691839));
#137403=DIRECTION('center_axis',(0.154510091262001,-0.475533164204444,-0.866022425483265));
#137404=DIRECTION('ref_axis',(-1.76891705781139E-15,0.876548714628816,-0.481313152617472));
#137405=DIRECTION('center_axis',(0.163755599459163,-0.503987842609615,-0.848045021297499));
#137406=DIRECTION('ref_axis',(0.266156471021525,-0.805199544416117,0.529919264233191));
#137407=DIRECTION('center_axis',(-0.163755570286403,0.503987822791173,0.848045038708669));
#137408=DIRECTION('ref_axis',(-1.1219235501908E-15,-0.859649495083722,0.510884278092703));
#137409=DIRECTION('center_axis',(0.154510105545767,-0.475533174128097,-0.866022417485768));
#137410=DIRECTION('ref_axis',(0.271938812468096,-0.822222161142252,0.500000000000006));
#137411=DIRECTION('center_axis',(0.267587483540088,-0.823661100222747,-0.499979330205296));
#137412=DIRECTION('ref_axis',(-0.153585232136767,0.475806237445614,-0.866036951219371));
#137413=DIRECTION('center_axis',(0.950981553003154,0.309247612517397,2.15946453637257E-15));
#137414=DIRECTION('ref_axis',(0.309247612517397,-0.950981553003154,-6.82961998416078E-15));
#137415=DIRECTION('center_axis',(-0.309016994374957,0.95105651629515,6.59767734033506E-15));
#137416=DIRECTION('ref_axis',(0.95105651629515,0.309016994374957,3.41480999208033E-15));
#137417=DIRECTION('center_axis',(0.309016994374964,-0.951056516295148,-6.64119215765934E-15));
#137418=DIRECTION('ref_axis',(-0.951056516295148,-0.309016994374964,-3.41480999208031E-15));
#137419=DIRECTION('center_axis',(-9.73020895656121E-17,-7.11688751458844E-15,
1.));
#137420=DIRECTION('ref_axis',(0.,-1.,-7.11547567313622E-15));
#137421=DIRECTION('center_axis',(0.951131423661011,0.308786358061005,2.15624361371867E-15));
#137422=DIRECTION('ref_axis',(0.308786358061005,-0.95113142366101,-6.82961998416062E-15));
#137423=DIRECTION('center_axis',(0.16375573087775,-0.503988317040604,0.848044713969301));
#137424=DIRECTION('ref_axis',(-1.79468021185938E-15,-0.859649189130452,
-0.510884792910649));
#137425=DIRECTION('center_axis',(0.163755570286399,-0.503987822791161,-0.848045038708677));
#137426=DIRECTION('ref_axis',(5.47345787009395E-16,0.85964949508373,-0.51088427809269));
#137427=DIRECTION('center_axis',(0.163755716972381,-0.503988355851568,0.848044693589256));
#137428=DIRECTION('ref_axis',(-0.266368911014076,0.805129291877831,0.52991926423322));
#137429=DIRECTION('center_axis',(0.163755751065492,-0.503988379171997,0.848044673146739));
#137430=DIRECTION('ref_axis',(2.0062615550087E-15,-0.859649150669469,-0.510884857627686));
#137431=DIRECTION('center_axis',(-0.163755599576498,0.503987842737942,0.848045021198578));
#137432=DIRECTION('ref_axis',(0.257959309144535,-0.807862963763176,0.529919264233196));
#137433=DIRECTION('center_axis',(0.1637555876299,-0.503987876168967,-0.84804500363759));
#137434=DIRECTION('ref_axis',(-9.1753207598515E-16,0.859649462041498,-0.510884333691847));
#137435=DIRECTION('center_axis',(0.95097670255072,0.309262527968972,2.15956869041424E-15));
#137436=DIRECTION('ref_axis',(0.309262527968972,-0.95097670255072,-6.82961998416085E-15));
#137437=DIRECTION('center_axis',(0.309016994374964,-0.951056516295148,-1.50830667185733E-14));
#137438=DIRECTION('ref_axis',(-0.951056516295148,-0.309016994374964,-3.41480999208024E-15));
#137439=DIRECTION('center_axis',(-9.73020895656121E-17,-7.11688751458844E-15,
1.));
#137440=DIRECTION('ref_axis',(0.,-1.,-7.11677149719761E-15));
#137441=DIRECTION('center_axis',(0.951136266645023,0.308771440182812,-6.95712478733879E-15));
#137442=DIRECTION('ref_axis',(0.308771440182812,-0.951136266645023,-6.82961998416072E-15));
#137443=DIRECTION('center_axis',(0.309016994374957,-0.95105651629515,-6.59767734033506E-15));
#137444=DIRECTION('ref_axis',(-0.95105651629515,-0.309016994374957,-3.41480999208025E-15));
#137445=DIRECTION('center_axis',(0.267642920194009,-0.823622990674208,0.500012436348234));
#137446=DIRECTION('ref_axis',(0.153571010716873,-0.47584571214317,-0.866017784403044));
#137447=DIRECTION('center_axis',(-0.163755751065471,0.503988379172021,-0.848044673146729));
#137448=DIRECTION('ref_axis',(-1.04962869149324E-15,0.859649150669455,0.510884857627709));
#137449=DIRECTION('center_axis',(-0.15451003561906,0.475533025685345,-0.866022511471577));
#137450=DIRECTION('ref_axis',(-0.263355672632978,0.825011387613578,0.49999999999995));
#137451=DIRECTION('center_axis',(0.154510049384271,-0.475533035318085,0.86602250372634));
#137452=DIRECTION('ref_axis',(8.3687170438306E-16,-0.876548788012466,-0.481313018974011));
#137453=DIRECTION('center_axis',(-0.163755716852405,0.5039883556864,-0.848044693710582));
#137454=DIRECTION('ref_axis',(-0.257746148189121,0.807930997355695,0.529919264233246));
#137455=DIRECTION('center_axis',(-0.163755730877757,0.503988317040565,-0.848044713969323));
#137456=DIRECTION('ref_axis',(9.15490063314203E-17,0.859649189130475,0.51088479291061));
#137457=DIRECTION('center_axis',(0.309016994374964,-0.951056516295148,-6.64119215765934E-15));
#137458=DIRECTION('ref_axis',(-0.951056516295148,-0.309016994374964,-3.41480999208031E-15));
#137459=DIRECTION('center_axis',(-0.309016994374964,0.951056516295148,6.64119215765934E-15));
#137460=DIRECTION('ref_axis',(0.951056516295148,0.309016994374964,3.41480999208031E-15));
#137461=DIRECTION('center_axis',(0.309016994374957,-0.95105651629515,-6.59767734033506E-15));
#137462=DIRECTION('ref_axis',(-0.95105651629515,-0.309016994374957,-3.41480999208025E-15));
#137463=DIRECTION('center_axis',(0.309016994374964,-0.951056516295148,-2.35249412794872E-14));
#137464=DIRECTION('ref_axis',(-0.951056516295148,-0.309016994374964,-3.41480999208017E-15));
#137465=DIRECTION('center_axis',(0.309016994374957,-0.95105651629515,-6.59767734033506E-15));
#137466=DIRECTION('ref_axis',(-0.95105651629515,-0.309016994374957,-3.41480999208025E-15));
#137467=DIRECTION('center_axis',(-0.267653025932585,0.823639804208793,0.499979330204792));
#137468=DIRECTION('ref_axis',(0.155418826429222,-0.475210466544568,0.866036951219668));
#137469=DIRECTION('center_axis',(0.154510091261982,-0.475533164204414,-0.866022425483285));
#137470=DIRECTION('ref_axis',(8.44054174721563E-16,0.876548714628834,-0.48131315261744));
#137471=DIRECTION('center_axis',(0.154510094034416,-0.475533172737053,-0.866022420303371));
#137472=DIRECTION('ref_axis',(0.951056516293818,0.309016994379058,-2.46959058042575E-12));
#137473=DIRECTION('center_axis',(-0.203370361063309,0.456777309670355,-0.866022508720929));
#137474=DIRECTION('ref_axis',(-0.913545457642283,-0.406736643076513,-4.37095680000764E-13));
#137475=DIRECTION('center_axis',(-0.352213899942317,0.791159233140904,-0.500012436348658));
#137476=DIRECTION('ref_axis',(-0.20427742789601,0.456381342245913,0.866017784402843));
#137477=DIRECTION('center_axis',(0.203370364581912,-0.456777317573279,0.866022503726306));
#137478=DIRECTION('ref_axis',(8.71792903940306E-16,-0.884507036382095,-0.46652685087845));
#137479=DIRECTION('center_axis',(0.406736643075807,-0.913545457642598,-6.37925383508808E-15));
#137480=DIRECTION('ref_axis',(-0.913545457642598,-0.406736643075807,-3.4148099920803E-15));
#137481=DIRECTION('center_axis',(-0.40673664307581,0.913545457642596,6.32197843909135E-15));
#137482=DIRECTION('ref_axis',(0.913545457642596,0.40673664307581,3.41480999208033E-15));
#137483=DIRECTION('center_axis',(-0.406736643075807,0.913545457642598,6.37925383508808E-15));
#137484=DIRECTION('ref_axis',(0.913545457642598,0.406736643075807,3.4148099920803E-15));
#137485=DIRECTION('center_axis',(-0.40673664307581,0.913545457642596,6.32197843909135E-15));
#137486=DIRECTION('ref_axis',(0.913545457642596,0.40673664307581,3.41480999208033E-15));
#137487=DIRECTION('center_axis',(0.406736643075817,-0.913545457642594,-6.37925383508805E-15));
#137488=DIRECTION('ref_axis',(-0.913545457642593,-0.406736643075817,-3.41480999208037E-15));
#137489=DIRECTION('center_axis',(-0.215539595588313,0.484109857923779,0.848045003637569));
#137490=DIRECTION('ref_axis',(-7.52396283484213E-16,-0.868458021515989,
0.495762710240023));
#137491=DIRECTION('center_axis',(0.20337041970248,-0.456777441376077,-0.866022425483291));
#137492=DIRECTION('ref_axis',(2.06048551024826E-15,0.884506966812056,-0.466526982779063));
#137493=DIRECTION('center_axis',(0.215539603854002,-0.484109823307635,-0.84804502129752));
#137494=DIRECTION('ref_axis',(0.348864709048125,-0.772967650148034,0.529919264233141));
#137495=DIRECTION('center_axis',(-0.21553957276031,0.484109806651245,0.848045038708674));
#137496=DIRECTION('ref_axis',(-2.70827771329659E-15,-0.868458052949983,
0.495762655175159));
#137497=DIRECTION('center_axis',(0.203370434941407,-0.456777449754108,-0.866022417485758));
#137498=DIRECTION('ref_axis',(0.356394722166398,-0.789292595943951,0.499999999999994));
#137499=DIRECTION('center_axis',(0.352217640366812,-0.791178490090451,-0.499979330205389));
#137500=DIRECTION('ref_axis',(-0.202479170973359,0.457145692799023,-0.866036951219313));
#137501=DIRECTION('center_axis',(0.913446798847318,0.406958162070241,2.77957517046168E-14));
#137502=DIRECTION('ref_axis',(0.406958162070241,-0.913446798847317,-6.82961998416E-15));
#137503=DIRECTION('center_axis',(-0.40673664307581,0.913545457642596,6.32197843909135E-15));
#137504=DIRECTION('ref_axis',(0.913545457642596,0.40673664307581,3.41480999208033E-15));
#137505=DIRECTION('center_axis',(0.406736643075817,-0.913545457642594,-6.37925383508805E-15));
#137506=DIRECTION('ref_axis',(-0.913545457642593,-0.406736643075817,-3.41480999208037E-15));
#137507=DIRECTION('center_axis',(-8.35415108931894E-17,-7.11160532333482E-15,
1.));
#137508=DIRECTION('ref_axis',(0.,-1.,-7.10842366553152E-15));
#137509=DIRECTION('center_axis',(0.913644062717548,0.406515100163541,2.8386797723579E-15));
#137510=DIRECTION('ref_axis',(0.406515100163541,-0.913644062717548,-6.82961998416062E-15));
#137511=DIRECTION('center_axis',(0.215539784135082,-0.484110281406718,0.848044713969323));
#137512=DIRECTION('ref_axis',(1.68888390132495E-15,-0.868457761888286,-0.495763165045559));
#137513=DIRECTION('center_axis',(0.215539572760321,-0.484109806651269,-0.848045038708658));
#137514=DIRECTION('ref_axis',(-1.90731993212003E-15,0.868458052949969,-0.495762655175185));
#137515=DIRECTION('center_axis',(0.215539774370431,-0.484110321455134,0.848044693589289));
#137516=DIRECTION('ref_axis',(-0.349068641859116,0.772875576444986,0.529919264233206));
#137517=DIRECTION('center_axis',(0.215539810706709,-0.484110341087605,0.848044673146739));
#137518=DIRECTION('ref_axis',(1.28899452946971E-15,-0.868457725299272,-0.4957632291407));
#137519=DIRECTION('center_axis',(-0.215539603976693,0.484109823426323,0.848045021198583));
#137520=DIRECTION('ref_axis',(0.340990855195057,-0.776473315747487,0.529919264233192));
#137521=DIRECTION('center_axis',(0.215539595588318,-0.484109857923791,-0.848045003637562));
#137522=DIRECTION('ref_axis',(1.78938953355032E-15,0.868458021515983,-0.495762710240035));
#137523=DIRECTION('center_axis',(0.913440415876953,0.406972488803039,5.55993783434714E-15));
#137524=DIRECTION('ref_axis',(0.406972488803039,-0.913440415876953,-6.82961998416052E-15));
#137525=DIRECTION('center_axis',(0.406736643075807,-0.913545457642598,-1.74906806584517E-14));
#137526=DIRECTION('ref_axis',(-0.913545457642598,-0.406736643075807,-3.4148099920803E-15));
#137527=DIRECTION('center_axis',(-8.35415108931894E-17,-7.11160532333482E-15,
1.));
#137528=DIRECTION('ref_axis',(0.,-1.,-7.10926435426808E-15));
#137529=DIRECTION('center_axis',(0.913650438514062,0.40650077023674,2.83857970701388E-15));
#137530=DIRECTION('ref_axis',(0.40650077023674,-0.913650438514061,-6.8296199841608E-15));
#137531=DIRECTION('center_axis',(0.40673664307581,-0.913545457642596,-6.32197843909135E-15));
#137532=DIRECTION('ref_axis',(-0.913545457642596,-0.40673664307581,-3.41480999208034E-15));
#137533=DIRECTION('center_axis',(0.352268789801391,-0.791134794600527,0.500012436349583));
#137534=DIRECTION('ref_axis',(0.202469153669914,-0.457186437803249,-0.86601778440224));
#137535=DIRECTION('center_axis',(-0.215539810706676,0.484110341087625,-0.848044673146736));
#137536=DIRECTION('ref_axis',(1.37118570194245E-16,0.868457725299263,0.495763229140716));
#137537=DIRECTION('center_axis',(-0.203370349886521,0.456777309431526,-0.866022511471572));
#137538=DIRECTION('ref_axis',(-0.348150155226398,0.79296372515764,0.499999999999954));
#137539=DIRECTION('center_axis',(0.203370364581896,-0.456777317573244,0.866022503726329));
#137540=DIRECTION('ref_axis',(-2.3251588633511E-15,-0.884507036382115,-0.466526850878411));
#137541=DIRECTION('center_axis',(-0.215539774219281,0.484110321309935,-0.848044693710592));
#137542=DIRECTION('ref_axis',(-0.340785973386751,0.776563258039779,0.529919264233231));
#137543=DIRECTION('center_axis',(-0.215539784135111,0.484110281406703,-0.848044713969324));
#137544=DIRECTION('ref_axis',(-2.77729088551537E-15,0.868457761888292,0.495763165045546));
#137545=DIRECTION('center_axis',(0.406736643075807,-0.913545457642598,-6.37925383508808E-15));
#137546=DIRECTION('ref_axis',(-0.913545457642598,-0.406736643075807,-3.4148099920803E-15));
#137547=DIRECTION('center_axis',(-0.406736643075817,0.913545457642594,6.37925383508805E-15));
#137548=DIRECTION('ref_axis',(0.913545457642593,0.406736643075817,3.41480999208037E-15));
#137549=DIRECTION('center_axis',(0.40673664307581,-0.913545457642596,-6.32197843909135E-15));
#137550=DIRECTION('ref_axis',(-0.913545457642596,-0.40673664307581,-3.41480999208034E-15));
#137551=DIRECTION('center_axis',(0.406736643075807,-0.913545457642598,4.73217298827553E-15));
#137552=DIRECTION('ref_axis',(-0.913545457642598,-0.406736643075807,-3.4148099920803E-15));
#137553=DIRECTION('center_axis',(0.40673664307581,-0.913545457642596,-6.32197843909135E-15));
#137554=DIRECTION('ref_axis',(-0.913545457642596,-0.40673664307581,-3.41480999208034E-15));
#137555=DIRECTION('center_axis',(-0.352280597670873,0.791150459692824,0.499979330205246));
#137556=DIRECTION('ref_axis',(0.204240445635154,-0.456361522796734,0.866036951219404));
#137557=DIRECTION('center_axis',(0.203370419702468,-0.456777441376063,-0.866022425483301));
#137558=DIRECTION('ref_axis',(1.64733859252707E-15,0.884506966812064,-0.466526982779048));
#137559=DIRECTION('center_axis',(0.203370423353679,-0.456777449576814,-0.866022420300448));
#137560=DIRECTION('ref_axis',(0.913545457642565,0.406736643075882,-5.24514813535308E-14));
#137561=DIRECTION('center_axis',(-0.250002507181017,0.433017044457075,-0.866022508721838));
#137562=DIRECTION('ref_axis',(-0.866025403783246,-0.500000000002066,-1.35499660801461E-12));
#137563=DIRECTION('center_axis',(-0.432983094186388,0.750008802378924,-0.50001243634825));
#137564=DIRECTION('ref_axis',(-0.250863215143673,0.432528431880919,0.866017784403076));
#137565=DIRECTION('center_axis',(0.250002511507219,-0.433017051950273,0.866022503726305));
#137566=DIRECTION('ref_axis',(-3.84832814192959E-16,-0.894424794863785,
-0.447218387740124));
#137567=DIRECTION('center_axis',(0.499999999999998,-0.86602540378444,-6.04742307255492E-15));
#137568=DIRECTION('ref_axis',(-0.86602540378444,-0.499999999999998,-3.41480999208026E-15));
#137569=DIRECTION('center_axis',(-0.50000000000001,0.866025403784433,5.97701461910992E-15));
#137570=DIRECTION('ref_axis',(0.866025403784433,0.50000000000001,3.41480999208033E-15));
#137571=DIRECTION('center_axis',(-0.50000000000001,0.866025403784433,6.04742307255487E-15));
#137572=DIRECTION('ref_axis',(0.866025403784433,0.50000000000001,3.41480999208034E-15));
#137573=DIRECTION('center_axis',(-0.50000000000001,0.866025403784433,5.97701461910992E-15));
#137574=DIRECTION('ref_axis',(0.866025403784433,0.50000000000001,3.41480999208033E-15));
#137575=DIRECTION('center_axis',(0.499999999999998,-0.86602540378444,-6.04742307255492E-15));
#137576=DIRECTION('ref_axis',(-0.86602540378444,-0.499999999999998,-3.41480999208026E-15));
#137577=DIRECTION('center_axis',(-0.264962106632877,0.458927830768622,0.848045003637587));
#137578=DIRECTION('ref_axis',(9.35163036390063E-16,-0.879478602053334,0.475938429348076));
#137579=DIRECTION('center_axis',(0.250002579266714,-0.433017169313211,-0.866022425483292));
#137580=DIRECTION('ref_axis',(-1.20805579666634E-15,0.894424730216419,-0.447218517033101));
#137581=DIRECTION('center_axis',(0.264962111232149,-0.458927795479733,-0.848045021297522));
#137582=DIRECTION('ref_axis',(0.427750712282121,-0.732266960566111,0.529919264233154));
#137583=DIRECTION('center_axis',(-0.264962078570518,0.45892778216319,0.848045038708656));
#137584=DIRECTION('ref_axis',(1.63750655949806E-15,-0.879478631391259,0.475938375135015));
#137585=DIRECTION('center_axis',(0.250002595299433,-0.433017176051559,-0.86602241748576));
#137586=DIRECTION('ref_axis',(0.436945896705958,-0.747715375896346,0.500000000000012));
#137587=DIRECTION('center_axis',(0.432988827019088,-0.750027562856358,-0.499979330205146));
#137588=DIRECTION('ref_axis',(-0.249154705663389,0.433476564266486,-0.866036951219469));
#137589=DIRECTION('center_axis',(0.865904130412325,0.500209992837883,3.49294771099265E-15));
#137590=DIRECTION('ref_axis',(0.500209992837883,-0.865904130412325,-6.82961998416073E-15));
#137591=DIRECTION('center_axis',(-0.50000000000001,0.866025403784433,5.97701461910992E-15));
#137592=DIRECTION('ref_axis',(0.866025403784433,0.50000000000001,3.41480999208033E-15));
#137593=DIRECTION('center_axis',(0.50000000000001,-0.866025403784433,-6.04742307255487E-15));
#137594=DIRECTION('ref_axis',(-0.866025403784433,-0.50000000000001,-3.41480999208034E-15));
#137595=DIRECTION('center_axis',(-7.04084534449538E-17,-7.10491369633528E-15,
1.));
#137596=DIRECTION('ref_axis',(0.,-1.,-7.10137165792683E-15));
#137597=DIRECTION('center_axis',(0.866146626230604,0.499789977760002,3.49001476137974E-15));
#137598=DIRECTION('ref_axis',(0.499789977760002,-0.866146626230603,-6.82961998416084E-15));
#137599=DIRECTION('center_axis',(0.264962338412816,-0.4589282322232,0.848044713969317));
#137600=DIRECTION('ref_axis',(-1.10874842197371E-15,-0.879478359737745,
-0.475938877118696));
#137601=DIRECTION('center_axis',(0.264962078570517,-0.458927782163174,-0.848045038708665));
#137602=DIRECTION('ref_axis',(-2.83667081435709E-15,0.879478631391268,-0.475938375134998));
#137603=DIRECTION('center_axis',(0.264962332884999,-0.45892827307457,0.848044693589278));
#137604=DIRECTION('ref_axis',(-0.427943903624788,0.732154074457648,0.529919264233188));
#137605=DIRECTION('center_axis',(0.264962371077225,-0.458928288799667,0.84804467314673));
#137606=DIRECTION('ref_axis',(-1.18836456492387E-15,-0.879478325588502,
-0.475938940222425));
#137607=DIRECTION('center_axis',(-0.264962111371018,0.458927795582427,0.84804502119856));
#137608=DIRECTION('ref_axis',(0.420286434057206,-0.736576463608523,0.529919264233185));
#137609=DIRECTION('center_axis',(0.264962106632849,-0.45892783076856,-0.848045003637629));
#137610=DIRECTION('ref_axis',(1.23612151778348E-15,0.879478602053371,-0.475938429348007));
#137611=DIRECTION('center_axis',(0.86589628485713,0.500223573885338,-2.01619277381436E-14));
#137612=DIRECTION('ref_axis',(0.500223573885338,-0.86589628485713,-6.82961998416088E-15));
#137613=DIRECTION('center_axis',(0.50000000000001,-0.866025403784433,-6.04742307255487E-15));
#137614=DIRECTION('ref_axis',(-0.866025403784433,-0.50000000000001,-3.41480999208034E-15));
#137615=DIRECTION('center_axis',(-7.04084534449538E-17,-7.10491369633528E-15,
1.));
#137616=DIRECTION('ref_axis',(0.,-1.,-7.10175721133855E-15));
#137617=DIRECTION('center_axis',(0.866154464985094,0.499776392786199,3.4899198980147E-15));
#137618=DIRECTION('ref_axis',(0.499776392786199,-0.866154464985094,-6.82961998416057E-15));
#137619=DIRECTION('center_axis',(0.50000000000001,-0.866025403784433,-5.97701461910992E-15));
#137620=DIRECTION('ref_axis',(-0.866025403784433,-0.50000000000001,-3.41480999208034E-15));
#137621=DIRECTION('center_axis',(0.433035128828067,-0.749978760164922,0.500012436347684));
#137622=DIRECTION('ref_axis',(0.249149002219344,-0.433518133173526,-0.866017784403326));
#137623=DIRECTION('center_axis',(-0.264962371077261,0.458928288799635,-0.848044673146736));
#137624=DIRECTION('ref_axis',(-7.08699178131369E-16,0.879478325588517,0.475938940222397));
#137625=DIRECTION('center_axis',(-0.250002496036225,0.433017045392176,-0.866022511471548));
#137626=DIRECTION('ref_axis',(-0.429130231857386,0.752228186194869,0.500000000000003));
#137627=DIRECTION('center_axis',(0.250002511507148,-0.433017051950198,0.866022503726363));
#137628=DIRECTION('ref_axis',(-1.69037570385203E-15,-0.894424794863828,
-0.447218387740038));
#137629=DIRECTION('center_axis',(-0.264962332727107,0.458928272941578,-0.848044693710579));
#137630=DIRECTION('ref_axis',(-0.42009207616774,0.736687329153668,0.529919264233253));
#137631=DIRECTION('center_axis',(-0.264962338412833,0.458928232223187,-0.848044713969319));
#137632=DIRECTION('ref_axis',(7.6134706593656E-16,0.879478359737751,0.475938877118685));
#137633=DIRECTION('center_axis',(0.50000000000001,-0.866025403784433,-1.9706663040877E-14));
#137634=DIRECTION('ref_axis',(-0.866025403784433,-0.50000000000001,-3.41480999208034E-15));
#137635=DIRECTION('center_axis',(-0.500000000000034,0.866025403784419,6.04742307255478E-15));
#137636=DIRECTION('ref_axis',(0.866025403784419,0.500000000000034,3.4148099920805E-15));
#137637=DIRECTION('center_axis',(0.50000000000001,-0.866025403784433,-5.97701461910992E-15));
#137638=DIRECTION('ref_axis',(-0.866025403784433,-0.50000000000001,-3.41480999208034E-15));
#137639=DIRECTION('center_axis',(0.50000000000001,-0.866025403784433,-3.97051783400485E-14));
#137640=DIRECTION('ref_axis',(-0.866025403784433,-0.50000000000001,-3.41480999208034E-15));
#137641=DIRECTION('center_axis',(0.50000000000001,-0.866025403784433,-5.97701461910992E-15));
#137642=DIRECTION('ref_axis',(-0.866025403784433,-0.50000000000001,-3.41480999208034E-15));
#137643=DIRECTION('center_axis',(-0.433048509462458,0.749993105181527,0.499979330205273));
#137644=DIRECTION('ref_axis',(0.25082436377922,-0.432512586703996,0.866036951219385));
#137645=DIRECTION('center_axis',(0.250002579266705,-0.433017169313181,-0.86602242548331));
#137646=DIRECTION('ref_axis',(-2.67459257803907E-15,0.894424730216435,-0.447218517033068));
#137647=DIRECTION('center_axis',(0.250002583751534,-0.433017177081167,-0.866022420304587));
#137648=DIRECTION('ref_axis',(0.866025403782456,0.500000000003435,-2.2860103956705E-12));
#137649=DIRECTION('center_axis',(-0.293895573515241,0.404512553892875,-0.866022508720883));
#137650=DIRECTION('ref_axis',(-0.809016994377429,-0.587785252289058,2.43025198077899E-12));
#137651=DIRECTION('center_axis',(-0.509008435042384,0.700641118228627,-0.500012436348379));
#137652=DIRECTION('ref_axis',(-0.294700492557513,0.403936649468912,0.866017784402947));
#137653=DIRECTION('center_axis',(0.293895578599988,-0.404512560891486,0.866022503726312));
#137654=DIRECTION('ref_axis',(-2.42787896315404E-15,-0.906035256115475,
-0.42320221487578));
#137655=DIRECTION('center_axis',(0.587785252292496,-0.809016994374931,-5.64933547733406E-15));
#137656=DIRECTION('ref_axis',(-0.809016994374931,-0.587785252292496,-3.41480999208037E-15));
#137657=DIRECTION('center_axis',(-0.587785252292482,0.809016994374941,5.5665653761908E-15));
#137658=DIRECTION('ref_axis',(0.809016994374941,0.587785252292482,3.41480999208033E-15));
#137659=DIRECTION('center_axis',(-0.587785252292496,0.809016994374931,3.77641347209492E-14));
#137660=DIRECTION('ref_axis',(0.809016994374931,0.587785252292496,3.41480999208037E-15));
#137661=DIRECTION('center_axis',(-0.587785252292482,0.809016994374941,5.5665653761908E-15));
#137662=DIRECTION('ref_axis',(0.809016994374941,0.587785252292482,3.41480999208033E-15));
#137663=DIRECTION('center_axis',(0.58778525229247,-0.80901699437495,-5.6493354773342E-15));
#137664=DIRECTION('ref_axis',(-0.80901699437495,-0.58778525229247,-3.41480999208022E-15));
#137665=DIRECTION('center_axis',(-0.31148163739031,0.42871769426275,0.848045003637591));
#137666=DIRECTION('ref_axis',(1.10162827415622E-15,-0.892442058026276,0.451162025292273));
#137667=DIRECTION('center_axis',(0.293895658256118,-0.404512670528665,-0.866022425483296));
#137668=DIRECTION('ref_axis',(-1.88316153394377E-15,0.906035197473502,-0.423202340422584));
#137669=DIRECTION('center_axis',(0.311481638275178,-0.428717658686835,-0.848045021297507));
#137670=DIRECTION('ref_axis',(0.501950189207944,-0.683543400925387,0.529919264233208));
#137671=DIRECTION('center_axis',(-0.311481604401037,0.428717648856911,0.848045038708652));
#137672=DIRECTION('ref_axis',(1.88777093301588E-15,-0.89244208477774,0.451161972375289));
#137673=DIRECTION('center_axis',(0.293895674908356,-0.404512675552017,-0.866022417485778));
#137674=DIRECTION('ref_axis',(0.512709800578015,-0.697946029712376,0.499999999999983));
#137675=DIRECTION('center_axis',(0.509016097474398,-0.700659176689513,-0.499979330205468));
#137676=DIRECTION('ref_axis',(-0.293100449228649,0.405058175802929,-0.866036951219269));
#137677=DIRECTION('center_axis',(0.808874435122379,0.587981418248444,4.10585229880193E-15));
#137678=DIRECTION('ref_axis',(0.587981418248444,-0.808874435122379,-6.82961998416087E-15));
#137679=DIRECTION('center_axis',(-0.587785252292482,0.809016994374941,5.5665653761908E-15));
#137680=DIRECTION('ref_axis',(0.809016994374941,0.587785252292482,3.41480999208033E-15));
#137681=DIRECTION('center_axis',(0.58778525229247,-0.80901699437495,-5.6493354773342E-15));
#137682=DIRECTION('ref_axis',(-0.80901699437495,-0.58778525229247,-3.41480999208022E-15));
#137683=DIRECTION('center_axis',(-5.80468057465775E-17,-7.09688594845552E-15,
1.));
#137684=DIRECTION('ref_axis',(0.,-1.,-7.09431965032213E-15));
#137685=DIRECTION('center_axis',(0.809159506053906,0.587589051772239,4.10311241834261E-15));
#137686=DIRECTION('ref_axis',(0.587589051772239,-0.809159506053906,-6.82961998416078E-15));
#137687=DIRECTION('center_axis',(0.3114819098639,-0.428718069290563,0.848044713969322));
#137688=DIRECTION('ref_axis',(2.56903958782145E-15,-0.892441837073384,-0.451162462358166));
#137689=DIRECTION('center_axis',(0.311481604401026,-0.428717648856896,-0.848045038708663));
#137690=DIRECTION('ref_axis',(-3.17710353883337E-15,0.892442084777749,-0.451161972375272));
#137691=DIRECTION('center_axis',(0.311481908636171,-0.428718110496195,0.848044693589283));
#137692=DIRECTION('ref_axis',(-0.502130522419991,0.683410939222361,0.529919264233183));
#137693=DIRECTION('center_axis',(0.311481948263223,-0.428718122142737,0.848044673146735));
#137694=DIRECTION('ref_axis',(-2.52135914302017E-15,-0.892441805934762,
-0.451162523953289));
#137695=DIRECTION('center_axis',(-0.311481638421796,0.428717658776018,0.84804502119857));
#137696=DIRECTION('ref_axis',(0.494977266825156,-0.688609525580972,0.529919264233192));
#137697=DIRECTION('center_axis',(0.311481637390356,-0.428717694262813,-0.848045003637543));
#137698=DIRECTION('ref_axis',(-3.15651889012676E-15,0.892442058026239,-0.451162025292347));
#137699=DIRECTION('center_axis',(0.808865212939996,0.58799410481359,3.62321511990407E-14));
#137700=DIRECTION('ref_axis',(0.58799410481359,-0.808865212939996,-6.82961998416104E-15));
#137701=DIRECTION('center_axis',(0.587785252292496,-0.809016994374931,2.64654637662811E-14));
#137702=DIRECTION('ref_axis',(-0.809016994374931,-0.587785252292496,-3.41480999208037E-15));
#137703=DIRECTION('center_axis',(-5.80468057465775E-17,-7.09688594845552E-15,
1.));
#137704=DIRECTION('ref_axis',(0.,-1.,-7.09425006840901E-15));
#137705=DIRECTION('center_axis',(0.80916872188328,0.587576360591353,3.62064098324204E-14));
#137706=DIRECTION('ref_axis',(0.587576360591353,-0.80916872188328,-6.82961998416123E-15));
#137707=DIRECTION('center_axis',(0.587785252292482,-0.809016994374941,-5.5665653761908E-15));
#137708=DIRECTION('ref_axis',(-0.809016994374941,-0.587785252292482,-3.41480999208029E-15));
#137709=DIRECTION('center_axis',(0.509057044368145,-0.700605801485404,0.500012436349499));
#137710=DIRECTION('ref_axis',(0.293099122177626,-0.40510011315436,-0.866017784402278));
#137711=DIRECTION('center_axis',(-0.311481948263288,0.428718122142708,-0.848044673146725));
#137712=DIRECTION('ref_axis',(1.36579927504424E-15,0.892441805934771,0.451162523953269));
#137713=DIRECTION('center_axis',(-0.293895562539147,0.404512555978629,-0.866022511471518));
#137714=DIRECTION('ref_axis',(-0.505408667900667,0.703251077788578,0.500000000000076));
#137715=DIRECTION('center_axis',(0.293895578599968,-0.404512560891393,0.866022503726362));
#137716=DIRECTION('ref_axis',(2.61834824672012E-15,-0.906035256115521,-0.423202214875681));
#137717=DIRECTION('center_axis',(-0.311481908458697,0.428718110385103,-0.848044693710629));
#137718=DIRECTION('ref_axis',(-0.494795562240512,0.688740099734032,0.529919264233196));
#137719=DIRECTION('center_axis',(-0.311481909863969,0.428718069290501,-0.848044713969328));
#137720=DIRECTION('ref_axis',(9.41989347612634E-16,0.892441837073413,0.45116246235811));
#137721=DIRECTION('center_axis',(0.587785252292496,-0.809016994374931,-5.64933547733406E-15));
#137722=DIRECTION('ref_axis',(-0.809016994374931,-0.587785252292496,-3.41480999208037E-15));
#137723=DIRECTION('center_axis',(-0.587785252292496,0.809016994374931,5.64933547733406E-15));
#137724=DIRECTION('ref_axis',(0.809016994374931,0.587785252292496,3.41480999208037E-15));
#137725=DIRECTION('center_axis',(0.587785252292482,-0.809016994374941,-5.5665653761908E-15));
#137726=DIRECTION('ref_axis',(-0.809016994374941,-0.587785252292482,-3.41480999208029E-15));
#137727=DIRECTION('center_axis',(0.587785252292496,-0.809016994374931,3.85528935811342E-14));
#137728=DIRECTION('ref_axis',(-0.809016994374931,-0.587785252292496,-3.41480999208037E-15));
#137729=DIRECTION('center_axis',(0.587785252292482,-0.809016994374941,-5.5665653761908E-15));
#137730=DIRECTION('ref_axis',(-0.809016994374941,-0.587785252292482,-3.41480999208029E-15));
#137731=DIRECTION('center_axis',(-0.50907185116305,0.700618669263803,0.499979330205204));
#137732=DIRECTION('ref_axis',(0.294660197697693,-0.403924952206856,0.86603695121943));
#137733=DIRECTION('center_axis',(0.293895658256114,-0.40451267052866,-0.8660224254833));
#137734=DIRECTION('ref_axis',(-2.92311624756912E-15,0.906035197473505,-0.423202340422578));
#137735=DIRECTION('center_axis',(0.293895663531775,-0.404512677789947,-0.866022420301244));
#137736=DIRECTION('ref_axis',(0.809016994371858,0.587785252296726,-2.98536348044732E-12));
#137737=DIRECTION('center_axis',(-0.334568658444528,0.371576139138116,-0.866022508720091));
#137738=DIRECTION('ref_axis',(-0.743144825479581,-0.669130606356429,1.87514046718231E-12));
#137739=DIRECTION('center_axis',(-0.579456972967815,0.64359706336816,-0.500012436348195));
#137740=DIRECTION('ref_axis',(-0.335308969634739,0.370919252641439,0.866017784403072));
#137741=DIRECTION('center_axis',(0.334568664232119,-0.371576145565826,0.866022503726306));
#137742=DIRECTION('ref_axis',(3.65930929999324E-16,-0.918982183096522,-0.394299058014537));
#137743=DIRECTION('center_axis',(0.669130606358875,-0.743144825477379,-5.18935258042421E-15));
#137744=DIRECTION('ref_axis',(-0.743144825477379,-0.669130606358875,-3.41480999208015E-15));
#137745=DIRECTION('center_axis',(-0.669130606358867,0.743144825477386,5.09512767813144E-15));
#137746=DIRECTION('ref_axis',(0.743144825477386,0.669130606358867,3.41480999208033E-15));
#137747=DIRECTION('center_axis',(-0.669130606358845,0.743144825477406,-3.54138214292235E-14));
#137748=DIRECTION('ref_axis',(0.743144825477406,0.669130606358845,3.41480999208033E-15));
#137749=DIRECTION('center_axis',(-0.669130606358867,0.743144825477386,5.09512767813144E-15));
#137750=DIRECTION('ref_axis',(0.743144825477386,0.669130606358867,3.41480999208033E-15));
#137751=DIRECTION('center_axis',(0.669130606358845,-0.743144825477406,-5.1893525804244E-15));
#137752=DIRECTION('ref_axis',(-0.743144825477406,-0.669130606358845,-3.41480999208033E-15));
#137753=DIRECTION('center_axis',(-0.354588510146749,0.393810436983626,0.848045003637587));
#137754=DIRECTION('ref_axis',(-2.37537055868933E-15,-0.906978223357771,
0.421177518814551));
#137755=DIRECTION('center_axis',(0.334568754912034,-0.371576246276106,-0.866022425483295));
#137756=DIRECTION('ref_axis',(1.32125764084643E-15,0.91898213146365,-0.394299178353857));
#137757=DIRECTION('center_axis',(0.354588507311481,-0.393810401507025,-0.848045021297509));
#137758=DIRECTION('ref_axis',(0.570650194834968,-0.627330796732771,0.529919264233185));
#137759=DIRECTION('center_axis',(-0.354588472592004,0.393810395274856,0.848045038708635));
#137760=DIRECTION('ref_axis',(1.94126359720515E-15,-0.906978247051288,0.421177467792109));
#137761=DIRECTION('center_axis',(0.334568771994927,-0.371576249534259,-0.866022417485749));
#137762=DIRECTION('ref_axis',(0.582856348568798,-0.640529840782626,0.500000000000032));
#137763=DIRECTION('center_axis',(0.579466481046765,-0.643614221961121,-0.49997933020542));
#137764=DIRECTION('ref_axis',(-0.333834922954767,0.372201885189424,-0.866036951219302));
#137765=DIRECTION('center_axis',(0.742982542253377,0.669310796197633,8.18371867718752E-14));
#137766=DIRECTION('ref_axis',(0.669310796197633,-0.742982542253377,-6.82961998416045E-15));
#137767=DIRECTION('center_axis',(-0.669130606358867,0.743144825477386,5.09512767813144E-15));
#137768=DIRECTION('ref_axis',(0.743144825477386,0.669130606358867,3.41480999208033E-15));
#137769=DIRECTION('center_axis',(0.669130606358845,-0.743144825477406,-5.1893525804244E-15));
#137770=DIRECTION('ref_axis',(-0.743144825477406,-0.669130606358845,-3.41480999208033E-15));
#137771=DIRECTION('center_axis',(-4.65920045970846E-17,-7.08761003338124E-15,
1.));
#137772=DIRECTION('ref_axis',(0.,-1.,-7.08726764271744E-15));
#137773=DIRECTION('center_axis',(0.743307065001304,0.668950377172438,4.67125551701929E-15));
#137774=DIRECTION('ref_axis',(0.668950377172438,-0.743307065001304,-6.82961998416086E-15));
#137775=DIRECTION('center_axis',(0.354588820328836,-0.393810781475676,0.84804471396933));
#137776=DIRECTION('ref_axis',(-9.24151213041885E-16,-0.906978027661855,
-0.421177940232642));
#137777=DIRECTION('center_axis',(0.354588472592016,-0.39381039527487,-0.848045038708624));
#137778=DIRECTION('ref_axis',(-1.09907770159185E-15,0.90697824705128,-0.421177467792125));
#137779=DIRECTION('center_axis',(0.354588823405941,-0.393810822592156,0.848044693589247));
#137780=DIRECTION('ref_axis',(-0.570815694152314,0.627180210708223,0.529919264233149));
#137781=DIRECTION('center_axis',(0.354588864042302,-0.393810830024569,0.848044673146734));
#137782=DIRECTION('ref_axis',(-3.45243234032312E-15,-0.906978000082629,
-0.421177999622623));
#137783=DIRECTION('center_axis',(-0.35458850746671,0.393810401580338,0.848045021198559));
#137784=DIRECTION('ref_axis',(0.564245025061867,-0.633098037500908,0.529919264233177));
#137785=DIRECTION('center_axis',(0.354588510146734,-0.393810436983609,-0.848045003637601));
#137786=DIRECTION('ref_axis',(1.15170691571856E-15,0.90697822335778,-0.421177518814531));
#137787=DIRECTION('center_axis',(0.742972044483923,0.669322449283885,6.49863705058814E-16));
#137788=DIRECTION('ref_axis',(0.669322449283885,-0.742972044483923,-6.82961998416066E-15));
#137789=DIRECTION('center_axis',(0.669130606358845,-0.743144825477406,-4.57925265900746E-14));
#137790=DIRECTION('ref_axis',(-0.743144825477406,-0.669130606358845,-3.41480999208032E-15));
#137791=DIRECTION('center_axis',(-4.65920045970846E-17,-7.08761003338124E-15,
1.));
#137792=DIRECTION('ref_axis',(0.,-1.,-7.08674292547948E-15));
#137793=DIRECTION('center_axis',(0.743317556935059,0.668938718831625,4.6711741072605E-15));
#137794=DIRECTION('ref_axis',(0.668938718831625,-0.743317556935059,-6.82961998416081E-15));
#137795=DIRECTION('center_axis',(0.669130606358867,-0.743144825477386,-5.09512767813144E-15));
#137796=DIRECTION('ref_axis',(-0.743144825477386,-0.669130606358867,-3.41480999208029E-15));
#137797=DIRECTION('center_axis',(0.579501624400542,-0.643556859037129,0.500012436348735));
#137798=DIRECTION('ref_axis',(0.333837986832196,-0.372243731506654,-0.866017784402739));
#137799=DIRECTION('center_axis',(-0.354588864042398,0.393810830024473,-0.848044673146738));
#137800=DIRECTION('ref_axis',(-2.5025141110171E-15,0.906978000082668,0.421177999622539));
#137801=DIRECTION('center_axis',(-0.334568647735589,0.371576142367659,-0.866022511471583));
#137802=DIRECTION('ref_axis',(-0.576149740773897,0.646569003437538,0.49999999999996));
#137803=DIRECTION('center_axis',(0.334568664232095,-0.371576145565871,0.866022503726296));
#137804=DIRECTION('ref_axis',(-1.84625828909707E-15,-0.918982183096503,
-0.39429905801458));
#137805=DIRECTION('center_axis',(-0.354588823230568,0.39381082248875,-0.848044693710594));
#137806=DIRECTION('ref_axis',(-0.564077964602082,0.633246889644838,0.529919264233251));
#137807=DIRECTION('center_axis',(-0.354588820328848,0.393810781475689,-0.848044713969318));
#137808=DIRECTION('ref_axis',(1.80372274773434E-15,0.906978027661848,0.421177940232658));
#137809=DIRECTION('center_axis',(0.669130606358845,-0.743144825477406,-4.1748614670039E-14));
#137810=DIRECTION('ref_axis',(-0.743144825477406,-0.669130606358845,-3.41480999208033E-15));
#137811=DIRECTION('center_axis',(-0.669130606358872,0.743144825477382,5.18935258042423E-15));
#137812=DIRECTION('ref_axis',(0.743144825477382,0.669130606358872,3.41480999208052E-15));
#137813=DIRECTION('center_axis',(0.669130606358867,-0.743144825477386,-5.09512767813144E-15));
#137814=DIRECTION('ref_axis',(-0.743144825477386,-0.669130606358867,-3.41480999208029E-15));
#137815=DIRECTION('center_axis',(0.669130606358845,-0.743144825477406,-4.1748614670037E-14));
#137816=DIRECTION('ref_axis',(-0.743144825477406,-0.669130606358845,-3.41480999208033E-15));
#137817=DIRECTION('center_axis',(0.669130606358867,-0.743144825477386,-5.09512767813144E-15));
#137818=DIRECTION('ref_axis',(-0.743144825477386,-0.669130606358867,-3.41480999208029E-15));
#137819=DIRECTION('center_axis',(-0.579517695131704,0.643568108591944,0.499979330205385));
#137820=DIRECTION('ref_axis',(0.335267672838309,-0.370911831399768,0.86603695121932));
#137821=DIRECTION('center_axis',(0.33456875491201,-0.371576246276107,-0.866022425483304));
#137822=DIRECTION('ref_axis',(1.31994420604537E-15,0.918982131463651,-0.394299178353854));
#137823=DIRECTION('center_axis',(0.334568760915655,-0.371576252943814,-0.866022420303076));
#137824=DIRECTION('ref_axis',(0.74314482547369,0.669130606362972,-3.1907984490043E-12));
#137825=DIRECTION('center_axis',(-0.371576139135394,0.334568658442094,-0.866022508722199));
#137826=DIRECTION('ref_axis',(-0.669130606360631,-0.743144825475798,1.34625469437943E-12));
#137827=DIRECTION('center_axis',(-0.643556859037041,0.57950162440116,-0.500012436348132));
#137828=DIRECTION('ref_axis',(-0.372243731510656,0.333837986826846,0.866017784403081));
#137829=DIRECTION('center_axis',(0.371576145565853,-0.334568664232091,0.866022503726306));
#137830=DIRECTION('ref_axis',(-0.918982183096511,-1.05744342495379E-15,
0.394299058014561));
#137831=DIRECTION('center_axis',(0.743144825477379,-0.669130606358875,-4.67251405070161E-15));
#137832=DIRECTION('ref_axis',(-0.669130606358875,-0.743144825477379,-6.82961998416085E-15));
#137833=DIRECTION('center_axis',(-0.743144825477402,0.66913060635885,4.56786669500646E-15));
#137834=DIRECTION('ref_axis',(0.669130606358849,0.743144825477402,6.82961998416066E-15));
#137835=DIRECTION('center_axis',(-0.743144825477406,0.669130606358845,4.6725140507014E-15));
#137836=DIRECTION('ref_axis',(0.669130606358845,0.743144825477406,6.82961998416065E-15));
#137837=DIRECTION('center_axis',(-0.743144825477402,0.66913060635885,4.56786669500646E-15));
#137838=DIRECTION('ref_axis',(0.66913060635885,0.743144825477402,6.82961998416066E-15));
#137839=DIRECTION('center_axis',(0.743144825477382,-0.669130606358872,-4.67251405070159E-15));
#137840=DIRECTION('ref_axis',(-0.669130606358872,-0.743144825477382,-6.82961998416048E-15));
#137841=DIRECTION('center_axis',(-0.393810436983627,0.354588510146739,0.84804500363759));
#137842=DIRECTION('ref_axis',(-0.906978223357771,-2.42620968147434E-15,
-0.421177518814551));
#137843=DIRECTION('center_axis',(0.371576246276117,-0.334568754912008,-0.866022425483301));
#137844=DIRECTION('ref_axis',(0.918982131463646,9.92141015011441E-16,0.394299178353865));
#137845=DIRECTION('center_axis',(0.393810430453619,-0.354588475163049,-0.848045021297501));
#137846=DIRECTION('ref_axis',(0.633098037503659,-0.564245025058769,0.529919264233188));
#137847=DIRECTION('center_axis',(-0.393810395274859,0.354588472591995,0.848045038708638));
#137848=DIRECTION('ref_axis',(-0.906978247051287,2.6316557495518E-15,-0.421177467792111));
#137849=DIRECTION('center_axis',(0.37157626360364,-0.334568756369229,-0.866022417485775));
#137850=DIRECTION('ref_axis',(0.646617000436438,-0.576095872877601,0.499999999999978));
#137851=DIRECTION('center_axis',(0.64356810859173,-0.579517695132084,-0.49997933020522));
#137852=DIRECTION('ref_axis',(-0.370911831406173,0.335267672830955,-0.866036951219423));
#137853=DIRECTION('center_axis',(0.668950377172403,0.743307065001336,5.19048549296485E-15));
#137854=DIRECTION('ref_axis',(0.743307065001336,-0.668950377172402,-3.41480999208038E-15));
#137855=DIRECTION('center_axis',(-0.743144825477402,0.66913060635885,4.56786669500646E-15));
#137856=DIRECTION('ref_axis',(0.669130606358849,0.743144825477402,6.82961998416066E-15));
#137857=DIRECTION('center_axis',(0.743144825477409,-0.669130606358842,-4.67251405070138E-15));
#137858=DIRECTION('ref_axis',(-0.669130606358842,-0.743144825477409,-6.82961998416067E-15));
#137859=DIRECTION('center_axis',(-3.61695511949404E-17,-7.07718757997909E-15,
1.));
#137860=DIRECTION('ref_axis',(0.,-1.,-7.08021563511275E-15));
#137861=DIRECTION('center_axis',(0.669310796197601,0.742982542253406,5.18821936272799E-15));
#137862=DIRECTION('ref_axis',(0.742982542253406,-0.669310796197601,-3.41480999208024E-15));
#137863=DIRECTION('center_axis',(0.393810781475729,-0.354588820328862,0.848044713969294));
#137864=DIRECTION('ref_axis',(-0.906978027661826,2.76586647871208E-15,0.421177940232704));
#137865=DIRECTION('center_axis',(0.393810395274862,-0.354588472591998,-0.848045038708635));
#137866=DIRECTION('ref_axis',(0.906978247051285,-1.98629810325044E-15,0.421177467792115));
#137867=DIRECTION('center_axis',(0.393810788840124,-0.354588860891335,0.848044693589262));
#137868=DIRECTION('ref_axis',(-0.633246889658985,0.564077964586254,0.529919264233195));
#137869=DIRECTION('center_axis',(0.393810830024499,-0.354588864042367,0.848044673146739));
#137870=DIRECTION('ref_axis',(-0.906978000082658,2.87858588363672E-16,0.421177999622561));
#137871=DIRECTION('center_axis',(-0.393810430617737,0.354588475217419,0.848045021198555));
#137872=DIRECTION('ref_axis',(0.627330796736552,-0.570650194830793,0.529919264233205));
#137873=DIRECTION('center_axis',(0.39381043698369,-0.354588510146796,-0.848045003637538));
#137874=DIRECTION('ref_axis',(0.906978223357735,-7.84757798853097E-16,0.421177518814629));
#137875=DIRECTION('center_axis',(0.668938718831589,0.743317556935091,5.19055875774668E-15));
#137876=DIRECTION('ref_axis',(0.743317556935091,-0.668938718831589,-3.41480999208028E-15));
#137877=DIRECTION('center_axis',(0.743144825477406,-0.669130606358845,-4.6725140507014E-15));
#137878=DIRECTION('ref_axis',(-0.669130606358845,-0.743144825477406,-6.82961998416065E-15));
#137879=DIRECTION('center_axis',(-3.61695511949404E-17,-7.07718757997909E-15,
1.));
#137880=DIRECTION('ref_axis',(0.,-1.,-7.07923578254995E-15));
#137881=DIRECTION('center_axis',(0.669322449283883,0.742972044483925,5.18814605719551E-15));
#137882=DIRECTION('ref_axis',(0.742972044483925,-0.669322449283883,-3.41480999208044E-15));
#137883=DIRECTION('center_axis',(0.743144825477402,-0.66913060635885,-4.56786669500646E-15));
#137884=DIRECTION('ref_axis',(-0.66913060635885,-0.743144825477402,-6.82961998416062E-15));
#137885=DIRECTION('center_axis',(0.64359706336872,-0.579456972965919,0.500012436349672));
#137886=DIRECTION('ref_axis',(0.370919252638004,-0.33530896964076,-0.866017784402213));
#137887=DIRECTION('center_axis',(-0.393810830024549,0.354588864042324,-0.848044673146734));
#137888=DIRECTION('ref_axis',(0.906978000082637,1.97446543713211E-15,-0.421177999622606));
#137889=DIRECTION('center_axis',(-0.371576128832093,0.334568662768457,-0.866022511471545));
#137890=DIRECTION('ref_axis',(-0.640578396537782,0.582802983768183,0.499999999999987));
#137891=DIRECTION('center_axis',(0.371576145565796,-0.33456866423204,0.866022503726349));
#137892=DIRECTION('ref_axis',(-0.91898218309654,2.29774910071685E-15,0.394299058014495));
#137893=DIRECTION('center_axis',(-0.393810788650038,0.354588860812297,-0.848044693710581));
#137894=DIRECTION('ref_axis',(-0.627180210742338,0.57081569411471,0.529919264233278));
#137895=DIRECTION('center_axis',(-0.393810781475744,0.354588820328784,-0.848044713969319));
#137896=DIRECTION('ref_axis',(0.906978027661825,-2.63639073947388E-15,-0.421177940232707));
#137897=DIRECTION('center_axis',(0.743144825477406,-0.669130606358845,-8.7164259707347E-15));
#137898=DIRECTION('ref_axis',(-0.669130606358845,-0.743144825477406,-6.82961998416065E-15));
#137899=DIRECTION('center_axis',(-0.743144825477406,0.669130606358845,4.6725140507014E-15));
#137900=DIRECTION('ref_axis',(0.669130606358845,0.743144825477406,6.82961998416065E-15));
#137901=DIRECTION('center_axis',(0.743144825477402,-0.66913060635885,-4.56786669500646E-15));
#137902=DIRECTION('ref_axis',(-0.66913060635885,-0.743144825477402,-6.82961998416062E-15));
#137903=DIRECTION('center_axis',(0.743144825477406,-0.669130606358845,-8.71642597073447E-15));
#137904=DIRECTION('ref_axis',(-0.669130606358845,-0.743144825477406,-6.82961998416065E-15));
#137905=DIRECTION('center_axis',(0.743144825477402,-0.66913060635885,-4.56786669500646E-15));
#137906=DIRECTION('ref_axis',(-0.66913060635885,-0.743144825477402,-6.82961998416062E-15));
#137907=DIRECTION('center_axis',(-0.643614221961265,0.579466481046755,0.499979330205245));
#137908=DIRECTION('ref_axis',(0.372201885190247,-0.333834922953591,0.866036951219402));
#137909=DIRECTION('center_axis',(0.371576246276125,-0.334568754912015,-0.866022425483295));
#137910=DIRECTION('ref_axis',(0.918982131463643,2.05752676658029E-15,0.394299178353873));
#137911=DIRECTION('center_axis',(0.371576252947017,-0.334568760918514,-0.866022420300598));
#137912=DIRECTION('ref_axis',(0.669130606357726,0.743144825478414,-8.82933269452628E-13));
#137913=DIRECTION('center_axis',(-0.404512553894895,0.293895573516703,-0.866022508719443));
#137914=DIRECTION('ref_axis',(-0.587785252300532,-0.809016994369093,5.74780819192983E-12));
#137915=DIRECTION('center_axis',(-0.700605801486583,0.509057044367303,-0.500012436348706));
#137916=DIRECTION('ref_axis',(-0.405100113146689,0.293099122186841,0.866017784402747));
#137917=DIRECTION('center_axis',(0.404512560891477,-0.293895578600012,0.866022503726308));
#137918=DIRECTION('ref_axis',(-0.906035256115478,-2.30820235819247E-15,
0.423202214875774));
#137919=DIRECTION('center_axis',(0.80901699437495,-0.58778525229247,-4.10448247925272E-15));
#137920=DIRECTION('ref_axis',(-0.58778525229247,-0.80901699437495,-6.82961998416043E-15));
#137921=DIRECTION('center_axis',(-0.809016994374955,0.587785252292463,3.99055920848342E-15));
#137922=DIRECTION('ref_axis',(0.587785252292463,0.809016994374955,6.82961998416066E-15));
#137923=DIRECTION('center_axis',(-0.80901699437495,0.58778525229247,4.10448247925272E-15));
#137924=DIRECTION('ref_axis',(0.58778525229247,0.80901699437495,6.82961998416043E-15));
#137925=DIRECTION('center_axis',(-0.809016994374955,0.587785252292463,3.99055920848342E-15));
#137926=DIRECTION('ref_axis',(0.587785252292463,0.809016994374955,6.82961998416066E-15));
#137927=DIRECTION('center_axis',(0.80901699437495,-0.58778525229247,-4.10448247925272E-15));
#137928=DIRECTION('ref_axis',(-0.58778525229247,-0.80901699437495,-6.82961998416043E-15));
#137929=DIRECTION('center_axis',(-0.428717694262757,0.311481637390284,0.848045003637597));
#137930=DIRECTION('ref_axis',(-0.892442058026274,8.07292141989185E-16,-0.451162025292277));
#137931=DIRECTION('center_axis',(0.404512670528679,-0.29389565825609,-0.866022425483299));
#137932=DIRECTION('ref_axis',(0.906035197473497,-2.09617485499778E-15,0.423202340422594));
#137933=DIRECTION('center_axis',(0.428717684111651,-0.311481603280926,-0.848045021297505));
#137934=DIRECTION('ref_axis',(0.68860952557847,-0.494977266828602,0.529919264233224));
#137935=DIRECTION('center_axis',(-0.428717648856936,0.311481604401024,0.848045038708643));
#137936=DIRECTION('ref_axis',(-0.892442084777728,6.67310720912807E-18,-0.451161972375313));
#137937=DIRECTION('center_axis',(0.404512687917536,-0.293895657888627,-0.866022417485796));
#137938=DIRECTION('ref_axis',(0.703293181139598,-0.505350078027689,0.499999999999954));
#137939=DIRECTION('center_axis',(0.700618669263885,-0.509071851163053,-0.499979330205085));
#137940=DIRECTION('ref_axis',(-0.403924952202812,0.29466019770305,-0.866036951219493));
#137941=DIRECTION('center_axis',(0.587589051772177,0.809159506053951,-3.85596848322865E-14));
#137942=DIRECTION('ref_axis',(0.809159506053951,-0.587589051772177,-3.41480999208123E-15));
#137943=DIRECTION('center_axis',(-0.809016994374955,0.587785252292463,3.99055920848342E-15));
#137944=DIRECTION('ref_axis',(0.587785252292463,0.809016994374955,6.82961998416066E-15));
#137945=DIRECTION('center_axis',(0.80901699437495,-0.58778525229247,-4.10448247925272E-15));
#137946=DIRECTION('ref_axis',(-0.58778525229247,-0.80901699437495,-6.82961998416043E-15));
#137947=DIRECTION('center_axis',(-2.68936361206573E-17,-7.0657327788296E-15,
1.));
#137948=DIRECTION('ref_axis',(0.,-1.,-7.06611161990336E-15));
#137949=DIRECTION('center_axis',(0.587981418248456,0.808874435122371,5.64833999139408E-15));
#137950=DIRECTION('ref_axis',(0.808874435122371,-0.587981418248456,-3.41480999208034E-15));
#137951=DIRECTION('center_axis',(0.428718069290566,-0.311481909863969,0.848044713969295));
#137952=DIRECTION('ref_axis',(-0.892441837073378,9.13395690474326E-16,0.451162462358178));
#137953=DIRECTION('center_axis',(0.428717648856939,-0.311481604401026,-0.848045038708642));
#137954=DIRECTION('ref_axis',(0.892442084777727,-9.59323760580522E-17,0.451161972375316));
#137955=DIRECTION('center_axis',(0.428718080851877,-0.31148194943812,0.848044693589266));
#137956=DIRECTION('ref_axis',(-0.688740099740449,0.494795562231596,0.529919264233179));
#137957=DIRECTION('center_axis',(0.428718122142669,-0.311481948263306,0.848044673146739));
#137958=DIRECTION('ref_axis',(-0.89244180593479,1.4497682461611E-15,0.451162523953232));
#137959=DIRECTION('center_axis',(-0.428717684279575,0.311481603319163,0.848045021198569));
#137960=DIRECTION('ref_axis',(0.683543400920389,-0.501950189214795,0.529919264233165));
#137961=DIRECTION('center_axis',(0.42871769426279,-0.311481637390308,-0.848045003637572));
#137962=DIRECTION('ref_axis',(0.892442058026255,1.78135499927075E-15,0.451162025292313));
#137963=DIRECTION('center_axis',(0.587576360591332,0.809168721883295,-6.45673796727378E-15));
#137964=DIRECTION('ref_axis',(0.809168721883294,-0.587576360591332,-3.41480999208043E-15));
#137965=DIRECTION('center_axis',(0.80901699437495,-0.58778525229247,2.8010316764361E-14));
#137966=DIRECTION('ref_axis',(-0.58778525229247,-0.80901699437495,-6.82961998416043E-15));
#137967=DIRECTION('center_axis',(-2.68936361206573E-17,-7.0657327788296E-15,
1.));
#137968=DIRECTION('ref_axis',(0.,-1.,-7.06422149669088E-15));
#137969=DIRECTION('center_axis',(0.587994104813612,0.80886521293998,1.77160014651075E-14));
#137970=DIRECTION('ref_axis',(0.80886521293998,-0.587994104813612,-3.41480999208048E-15));
#137971=DIRECTION('center_axis',(0.809016994374955,-0.587785252292463,-3.99055920848342E-15));
#137972=DIRECTION('ref_axis',(-0.587785252292463,-0.809016994374955,-6.82961998416068E-15));
#137973=DIRECTION('center_axis',(0.700641118228849,-0.50900843504249,0.50001243634796));
#137974=DIRECTION('ref_axis',(0.40393664952349,-0.294700492481754,-0.86601778440327));
#137975=DIRECTION('center_axis',(-0.428718122142697,0.311481948263298,-0.848044673146727));
#137976=DIRECTION('ref_axis',(0.892441805934776,8.55497766242104E-16,-0.45116252395326));
#137977=DIRECTION('center_axis',(-0.404512544094918,0.293895578895568,-0.866022511471553));
#137978=DIRECTION('ref_axis',(-0.697988741330392,0.512651652660993,0.499999999999968));
#137979=DIRECTION('center_axis',(0.404512560891374,-0.293895578599945,0.866022503726379));
#137980=DIRECTION('ref_axis',(-0.906035256115532,-1.99991727152335E-15,
0.423202214875657));
#137981=DIRECTION('center_axis',(-0.428718080659361,0.311481949372824,-0.848044693710573));
#137982=DIRECTION('ref_axis',(-0.683410939245724,0.502130522388065,0.529919264233304));
#137983=DIRECTION('center_axis',(-0.428718069290593,0.311481909863882,-0.848044713969314));
#137984=DIRECTION('ref_axis',(0.89244183707337,-4.01305572582718E-16,-0.451162462358193));
#137985=DIRECTION('center_axis',(0.80901699437495,-0.58778525229247,2.80103167643593E-14));
#137986=DIRECTION('ref_axis',(-0.58778525229247,-0.80901699437495,-6.82961998416043E-15));
#137987=DIRECTION('center_axis',(-0.809016994374976,0.587785252292434,4.10448247925247E-15));
#137988=DIRECTION('ref_axis',(0.587785252292434,0.809016994374976,6.82961998416065E-15));
#137989=DIRECTION('center_axis',(0.809016994374955,-0.587785252292463,-3.99055920848342E-15));
#137990=DIRECTION('ref_axis',(-0.587785252292463,-0.809016994374955,-6.82961998416068E-15));
#137991=DIRECTION('center_axis',(0.80901699437495,-0.58778525229247,-4.10448247925272E-15));
#137992=DIRECTION('ref_axis',(-0.58778525229247,-0.80901699437495,-6.82961998416043E-15));
#137993=DIRECTION('center_axis',(0.809016994374955,-0.587785252292463,-3.99055920848342E-15));
#137994=DIRECTION('ref_axis',(-0.587785252292463,-0.809016994374955,-6.82961998416068E-15));
#137995=DIRECTION('center_axis',(-0.700659176689953,0.509016097474098,0.499979330205156));
#137996=DIRECTION('ref_axis',(0.405058175796856,-0.293100449236484,0.866036951219458));
#137997=DIRECTION('center_axis',(0.404512670528659,-0.293895658256083,-0.866022425483311));
#137998=DIRECTION('ref_axis',(0.906035197473507,-2.80279631697786E-15,0.423202340422572));
#137999=DIRECTION('center_axis',(0.404512677794142,-0.293895663534851,-0.866022420298241));
#138000=DIRECTION('ref_axis',(0.587785252294639,0.809016994373374,1.48175434825272E-12));
#138001=DIRECTION('center_axis',(-0.433017044458074,0.250002507181587,-0.866022508721173));
#138002=DIRECTION('ref_axis',(-0.500000000002247,-0.866025403783142,1.47738339837865E-12));
#138003=DIRECTION('center_axis',(-0.749978760163501,0.433035128829403,-0.500012436348657));
#138004=DIRECTION('ref_axis',(-0.433518133169102,0.249149002228967,0.866017784402773));
#138005=DIRECTION('center_axis',(0.43301705195027,-0.250002511507207,0.86602250372631));
#138006=DIRECTION('ref_axis',(-0.894424794863787,-7.00304685398516E-16,
0.44721838774012));
#138007=DIRECTION('center_axis',(0.866025403784433,-0.50000000000001,-3.4914813388432E-15));
#138008=DIRECTION('ref_axis',(-0.50000000000001,-0.866025403784433,-6.82961998416068E-15));
#138009=DIRECTION('center_axis',(-0.866025403784445,0.499999999999989,3.36953032019404E-15));
#138010=DIRECTION('ref_axis',(0.499999999999989,0.866025403784445,6.82961998416066E-15));
#138011=DIRECTION('center_axis',(-0.86602540378444,0.499999999999998,1.71507213071642E-14));
#138012=DIRECTION('ref_axis',(0.499999999999998,0.86602540378444,6.82961998416091E-15));
#138013=DIRECTION('center_axis',(-0.866025403784445,0.499999999999989,3.36953032019404E-15));
#138014=DIRECTION('ref_axis',(0.499999999999989,0.866025403784445,6.82961998416066E-15));
#138015=DIRECTION('center_axis',(0.866025403784463,-0.499999999999957,-3.49148133884283E-15));
#138016=DIRECTION('ref_axis',(-0.499999999999957,-0.866025403784463,-6.8296199841607E-15));
#138017=DIRECTION('center_axis',(-0.458927830768608,0.26496210663286,0.8480450036376));
#138018=DIRECTION('ref_axis',(-0.879478602053343,1.78405630805235E-15,-0.47593842934806));
#138019=DIRECTION('center_axis',(0.43301716931321,-0.250002579266712,-0.866022425483294));
#138020=DIRECTION('ref_axis',(0.89442473021642,-1.02528410709423E-15,0.447218517033099));
#138021=DIRECTION('center_axis',(0.458927817106631,-0.264962073773304,-0.84804502129751));
#138022=DIRECTION('ref_axis',(0.736576463600031,-0.420286434072047,0.529919264233217));
#138023=DIRECTION('center_axis',(-0.458927782163189,0.264962078570508,0.84804503870866));
#138024=DIRECTION('ref_axis',(-0.87947863139126,1.76485634666569E-15,-0.475938375135012));
#138025=DIRECTION('center_axis',(0.433017186567159,-0.250002577085787,-0.866022417485787));
#138026=DIRECTION('ref_axis',(0.752263934581057,-0.429067561962785,0.499999999999939));
#138027=DIRECTION('center_axis',(0.749993105181555,-0.433048509462383,-0.499979330205297));
#138028=DIRECTION('ref_axis',(-0.43251258670008,0.250824363786042,-0.866036951219365));
#138029=DIRECTION('center_axis',(0.499789977759954,0.866146626230631,6.04826956437238E-15));
#138030=DIRECTION('ref_axis',(0.866146626230631,-0.499789977759954,-3.41480999208016E-15));
#138031=DIRECTION('center_axis',(-0.866025403784445,0.499999999999989,3.36953032019404E-15));
#138032=DIRECTION('ref_axis',(0.499999999999989,0.866025403784445,6.82961998416066E-15));
#138033=DIRECTION('center_axis',(0.86602540378444,-0.499999999999998,-3.49148133884312E-15));
#138034=DIRECTION('ref_axis',(-0.499999999999998,-0.86602540378444,-6.82961998416073E-15));
#138035=DIRECTION('center_axis',(-1.88658882408992E-17,-7.05337113113122E-15,
1.));
#138036=DIRECTION('ref_axis',(0.,-1.,-7.05200760469397E-15));
#138037=DIRECTION('center_axis',(0.500209992837931,0.865904130412297,6.04657622512345E-15));
#138038=DIRECTION('ref_axis',(0.865904130412297,-0.500209992837931,-3.41480999208038E-15));
#138039=DIRECTION('center_axis',(0.458928232223227,-0.264962338412759,0.848044713969321));
#138040=DIRECTION('ref_axis',(-0.879478359737734,-3.02123578176224E-15,
0.475938877118716));
#138041=DIRECTION('center_axis',(0.458927782163212,-0.264962078570521,-0.848045038708643));
#138042=DIRECTION('ref_axis',(0.879478631391247,-3.81712923167341E-16,0.475938375135038));
#138043=DIRECTION('center_axis',(0.458928247861605,-0.264962376555123,0.848044693589282));
#138044=DIRECTION('ref_axis',(-0.736687329166148,0.420092076145952,0.529919264233176));
#138045=DIRECTION('center_axis',(0.458928288799633,-0.264962371077261,0.848044673146737));
#138046=DIRECTION('ref_axis',(-0.879478325588518,6.87163476984199E-16,0.475938940222395));
#138047=DIRECTION('center_axis',(-0.458927817275418,0.264962073797621,0.848045021198571));
#138048=DIRECTION('ref_axis',(0.732266960588852,-0.427750712242988,0.529919264233318));
#138049=DIRECTION('center_axis',(0.458927830768628,-0.264962106632871,-0.848045003637586));
#138050=DIRECTION('ref_axis',(0.879478602053331,-1.57823178879883E-16,0.475938429348081));
#138051=DIRECTION('center_axis',(0.499776392786184,0.866154464985103,2.97103476758322E-14));
#138052=DIRECTION('ref_axis',(0.866154464985103,-0.499776392786184,-3.4148099920807E-15));
#138053=DIRECTION('center_axis',(0.86602540378444,-0.499999999999998,-3.49148133884312E-15));
#138054=DIRECTION('ref_axis',(-0.499999999999998,-0.86602540378444,-6.82961998416073E-15));
#138055=DIRECTION('center_axis',(-1.88658882408992E-17,-7.05337113113122E-15,
1.));
#138056=DIRECTION('ref_axis',(0.,-1.,-7.05671435376135E-15));
#138057=DIRECTION('center_axis',(0.500223573885301,0.865896284857152,6.04652143990469E-15));
#138058=DIRECTION('ref_axis',(0.865896284857152,-0.500223573885301,-3.41480999208034E-15));
#138059=DIRECTION('center_axis',(0.866025403784445,-0.499999999999989,-3.36953032019404E-15));
#138060=DIRECTION('ref_axis',(-0.499999999999989,-0.866025403784445,-6.82961998416055E-15));
#138061=DIRECTION('center_axis',(0.750008802379763,-0.432983094187063,0.500012436346408));
#138062=DIRECTION('ref_axis',(0.432528431901353,-0.250863215104638,-0.866017784404178));
#138063=DIRECTION('center_axis',(-0.458928288799654,0.264962371077256,-0.848044673146728));
#138064=DIRECTION('ref_axis',(0.879478325588507,7.27534261071945E-16,-0.475938940222415));
#138065=DIRECTION('center_axis',(-0.433017035277113,0.250002513556067,-0.866022511471537));
#138066=DIRECTION('ref_axis',(-0.747751775423434,0.436883602749162,0.500000000000014));
#138067=DIRECTION('center_axis',(0.433017051950193,-0.250002511507147,0.866022503726365));
#138068=DIRECTION('ref_axis',(-0.894424794863831,-1.74682411385781E-15,
0.447218387740033));
#138069=DIRECTION('center_axis',(-0.45892824765206,0.264962376529661,-0.848044693710634));
#138070=DIRECTION('ref_axis',(-0.732154074452537,0.4279439036336,0.529919264233132));
#138071=DIRECTION('center_axis',(-0.458928232223214,0.264962338412759,-0.848044713969328));
#138072=DIRECTION('ref_axis',(0.879478359737742,2.18132396275747E-15,-0.475938877118703));
#138073=DIRECTION('center_axis',(0.86602540378444,-0.499999999999998,-3.71492366063374E-14));
#138074=DIRECTION('ref_axis',(-0.499999999999998,-0.86602540378444,-6.82961998416119E-15));
#138075=DIRECTION('center_axis',(-0.866025403784433,0.50000000000001,3.4914813388432E-15));
#138076=DIRECTION('ref_axis',(0.50000000000001,0.866025403784433,6.82961998416068E-15));
#138077=DIRECTION('center_axis',(0.866025403784445,-0.499999999999989,-3.36953032019404E-15));
#138078=DIRECTION('ref_axis',(-0.499999999999989,-0.866025403784445,-6.82961998416055E-15));
#138079=DIRECTION('center_axis',(0.86602540378444,-0.499999999999998,2.38269985977989E-14));
#138080=DIRECTION('ref_axis',(-0.499999999999998,-0.86602540378444,-6.82961998416036E-15));
#138081=DIRECTION('center_axis',(0.866025403784445,-0.499999999999989,-3.36953032019404E-15));
#138082=DIRECTION('ref_axis',(-0.499999999999989,-0.866025403784445,-6.82961998416055E-15));
#138083=DIRECTION('center_axis',(-0.750027562856428,0.43298882701908,0.499979330205047));
#138084=DIRECTION('ref_axis',(0.43347656427264,-0.24915470565252,0.866036951219516));
#138085=DIRECTION('center_axis',(0.433017169313169,-0.250002579266681,-0.866022425483323));
#138086=DIRECTION('ref_axis',(0.894424730216443,2.17074162788549E-15,0.447218517033052));
#138087=DIRECTION('center_axis',(0.433017177085757,-0.250002583754148,-0.866022420301537));
#138088=DIRECTION('ref_axis',(0.499999999999688,0.866025403784619,-1.44241573722197E-13));
#138089=DIRECTION('center_axis',(-0.45677730966968,0.203370361063029,-0.866022508721351));
#138090=DIRECTION('ref_axis',(-0.406736643071311,-0.9135454576446,-2.85423479040283E-12));
#138091=DIRECTION('center_axis',(-0.79113479460122,0.352268789800861,-0.500012436348859));
#138092=DIRECTION('ref_axis',(0.457186437780581,-0.202469153719109,-0.866017784402706));
#138093=DIRECTION('center_axis',(0.456777317573273,-0.203370364581924,0.866022503726307));
#138094=DIRECTION('ref_axis',(-0.884507036382098,8.12886901361279E-16,0.466526850878445));
#138095=DIRECTION('center_axis',(0.913545457642598,-0.406736643075807,-2.84022679824576E-15));
#138096=DIRECTION('ref_axis',(-0.406736643075807,-0.913545457642598,-6.8296199841606E-15));
#138097=DIRECTION('center_axis',(-0.913545457642606,0.406736643075789,2.71158415259707E-15));
#138098=DIRECTION('ref_axis',(0.406736643075789,0.913545457642606,6.82961998416066E-15));
#138099=DIRECTION('center_axis',(-0.913545457642598,0.406736643075807,1.39516536216094E-14));
#138100=DIRECTION('ref_axis',(0.406736643075807,0.913545457642598,6.8296199841606E-15));
#138101=DIRECTION('center_axis',(-0.913545457642606,0.406736643075789,2.71158415259707E-15));
#138102=DIRECTION('ref_axis',(0.406736643075789,0.913545457642606,6.82961998416066E-15));
#138103=DIRECTION('center_axis',(0.913545457642598,-0.406736643075807,-2.84022679824576E-15));
#138104=DIRECTION('ref_axis',(-0.406736643075807,-0.913545457642598,-6.8296199841606E-15));
#138105=DIRECTION('center_axis',(-0.484109857923765,0.215539595588298,0.848045003637581));
#138106=DIRECTION('ref_axis',(-0.868458021515998,4.63801329176873E-17,-0.495762710240007));
#138107=DIRECTION('center_axis',(0.456777441376074,-0.203370419702464,-0.866022425483296));
#138108=DIRECTION('ref_axis',(0.884506966812059,1.56015689162916E-15,0.466526982779058));
#138109=DIRECTION('center_axis',(0.484109840903269,-0.215539564333573,-0.848045021297516));
#138110=DIRECTION('ref_axis',(0.776473315755943,-0.340990855175849,0.52991926423316));
#138111=DIRECTION('center_axis',(-0.484109806651279,0.215539572760317,0.848045038708653));
#138112=DIRECTION('ref_axis',(-0.868458052949963,1.30155882390688E-15,-0.495762655175195));
#138113=DIRECTION('center_axis',(0.456777458308535,-0.203370415727759,-0.866022417485779));
#138114=DIRECTION('ref_axis',(0.792992726925666,-0.348084091913183,0.49999999999997));
#138115=DIRECTION('center_axis',(0.791150459692744,-0.352280597670873,-0.499979330205373));
#138116=DIRECTION('ref_axis',(0.456361522796686,-0.204240445635572,0.86603695121933));
#138117=DIRECTION('center_axis',(0.406515100163541,0.913644062717548,6.37994239064629E-15));
#138118=DIRECTION('ref_axis',(0.913644062717548,-0.406515100163541,-3.41480999208033E-15));
#138119=DIRECTION('center_axis',(-0.913545457642606,0.406736643075789,2.71158415259707E-15));
#138120=DIRECTION('ref_axis',(0.406736643075789,0.913545457642606,6.82961998416066E-15));
#138121=DIRECTION('center_axis',(0.913545457642618,-0.406736643075761,-2.84022679824544E-15));
#138122=DIRECTION('ref_axis',(-0.406736643075761,-0.913545457642618,-6.82961998416076E-15));
#138123=DIRECTION('center_axis',(-1.2174261241351E-17,-7.04023807368298E-15,
1.));
#138124=DIRECTION('ref_axis',(0.,-1.,-7.03790358948458E-15));
#138125=DIRECTION('center_axis',(0.406958162070199,0.913446798847336,6.37856490440294E-15));
#138126=DIRECTION('ref_axis',(0.913446798847336,-0.406958162070199,-3.4148099920803E-15));
#138127=DIRECTION('center_axis',(0.484110281406754,-0.215539784135097,0.848044713969298));
#138128=DIRECTION('ref_axis',(-0.868457761888264,-7.52957874888421E-16,
0.495763165045596));
#138129=DIRECTION('center_axis',(0.484109806651376,-0.215539572760309,-0.8480450387086));
#138130=DIRECTION('ref_axis',(0.868458052949907,-1.21988200561595E-15,0.495762655175294));
#138131=DIRECTION('center_axis',(0.484110300947392,-0.215539820431551,0.848044693589294));
#138132=DIRECTION('ref_axis',(-0.776563258037247,0.340785973392536,0.529919264233221));
#138133=DIRECTION('center_axis',(0.484110341087594,-0.215539810706751,0.848044673146734));
#138134=DIRECTION('ref_axis',(-0.868457725299276,1.07363447275437E-15,0.495763229140693));
#138135=DIRECTION('center_axis',(-0.484109841074222,0.215539564339001,0.848045021198548));
#138136=DIRECTION('ref_axis',(0.772967650155928,-0.348864709030508,0.529919264233224));
#138137=DIRECTION('center_axis',(0.484109857923745,-0.215539595588289,-0.848045003637595));
#138138=DIRECTION('ref_axis',(0.868458021516011,-1.65169124191511E-15,0.495762710239986));
#138139=DIRECTION('center_axis',(0.406500770236715,0.913650438514073,9.12956181436392E-15));
#138140=DIRECTION('ref_axis',(0.913650438514073,-0.406500770236715,-3.41480999208026E-15));
#138141=DIRECTION('center_axis',(0.913545457642598,-0.406736643075807,-5.27535733098856E-14));
#138142=DIRECTION('ref_axis',(-0.406736643075807,-0.913545457642598,-6.8296199841606E-15));
#138143=DIRECTION('center_axis',(-1.2174261241351E-17,-7.04023807368298E-15,
1.));
#138144=DIRECTION('ref_axis',(0.,-1.,-7.04170006790228E-15));
#138145=DIRECTION('center_axis',(0.406972488803016,0.913440415876963,9.09658446655107E-15));
#138146=DIRECTION('ref_axis',(0.913440415876963,-0.406972488803016,-3.41480999208023E-15));
#138147=DIRECTION('center_axis',(0.913545457642606,-0.406736643075789,-2.71158415259707E-15));
#138148=DIRECTION('ref_axis',(-0.406736643075789,-0.913545457642606,-6.82961998416066E-15));
#138149=DIRECTION('center_axis',(0.791159233141483,-0.35221389994137,0.500012436348408));
#138150=DIRECTION('ref_axis',(0.45638134222745,-0.204277427936816,-0.866017784402948));
#138151=DIRECTION('center_axis',(-0.484110341087625,0.21553981070667,-0.848044673146737));
#138152=DIRECTION('ref_axis',(0.868457725299263,1.08885966448668E-16,-0.495763229140716));
#138153=DIRECTION('center_axis',(-0.456777301207149,0.203370368358987,-0.866022511471523));
#138154=DIRECTION('ref_axis',(-0.789322284581999,0.356328964669224,0.500000000000013));
#138155=DIRECTION('center_axis',(0.456777317573189,-0.203370364581881,0.866022503726361));
#138156=DIRECTION('ref_axis',(-0.884507036382145,2.90703320888221E-16,0.466526850878355));
#138157=DIRECTION('center_axis',(-0.484110300735212,0.215539820430766,-0.848044693710618));
#138158=DIRECTION('ref_axis',(-0.77287557643843,0.349068641873687,0.529919264233171));
#138159=DIRECTION('center_axis',(-0.484110281406742,0.215539784135022,-0.848044713969325));
#138160=DIRECTION('ref_axis',(0.868457761888276,-5.66899354755573E-16,-0.495763165045576));
#138161=DIRECTION('center_axis',(0.913545457642598,-0.406736643075807,-1.39516536216094E-14));
#138162=DIRECTION('ref_axis',(-0.406736643075807,-0.913545457642598,-6.8296199841606E-15));
#138163=DIRECTION('center_axis',(-0.913545457642594,0.406736643075817,2.84022679824583E-15));
#138164=DIRECTION('ref_axis',(0.406736643075817,0.913545457642593,6.82961998416057E-15));
#138165=DIRECTION('center_axis',(0.913545457642606,-0.406736643075789,-2.71158415259707E-15));
#138166=DIRECTION('ref_axis',(-0.406736643075789,-0.913545457642606,-6.82961998416066E-15));
#138167=DIRECTION('center_axis',(0.913545457642598,-0.406736643075807,5.81845465367577E-14));
#138168=DIRECTION('ref_axis',(-0.406736643075807,-0.913545457642598,-6.8296199841606E-15));
#138169=DIRECTION('center_axis',(0.913545457642606,-0.406736643075789,-2.71158415259707E-15));
#138170=DIRECTION('ref_axis',(-0.406736643075789,-0.913545457642606,-6.82961998416066E-15));
#138171=DIRECTION('center_axis',(-0.791178490090691,0.352217640366613,0.499979330205149));
#138172=DIRECTION('ref_axis',(0.457145692800845,-0.202479170968668,0.866036951219448));
#138173=DIRECTION('center_axis',(0.45677744137607,-0.203370419702462,-0.866022425483298));
#138174=DIRECTION('ref_axis',(0.884506966812061,1.8264828060639E-15,0.466526982779054));
#138175=DIRECTION('center_axis',(0.456777449574815,-0.203370423352742,-0.866022420301723));
#138176=DIRECTION('ref_axis',(0.406736643081688,0.913545457639979,3.74590996000316E-12));
#138177=DIRECTION('center_axis',(-0.475533027088392,0.154510046710294,-0.866022508722339));
#138178=DIRECTION('ref_axis',(-0.309016994372082,-0.951056516296084,-1.77460846079056E-12));
#138179=DIRECTION('center_axis',(-0.823622990674915,0.267642920194302,-0.500012436346914));
#138180=DIRECTION('ref_axis',(0.475845712136155,-0.153571010734221,-0.866017784403823));
#138181=DIRECTION('center_axis',(0.475533035318122,-0.1545100493843,0.866022503726315));
#138182=DIRECTION('ref_axis',(-0.876548788012444,-1.07841122773221E-15,
0.481313018974051));
#138183=DIRECTION('center_axis',(0.951056516295165,-0.309016994374914,5.82468571404663E-14));
#138184=DIRECTION('ref_axis',(-0.309016994374914,-0.951056516295164,-6.82961998416066E-15));
#138185=DIRECTION('center_axis',(-0.951056516295158,0.309016994374935,2.02392930158878E-15));
#138186=DIRECTION('ref_axis',(0.309016994374935,0.951056516295158,6.82961998416066E-15));
#138187=DIRECTION('center_axis',(-0.951056516295165,0.309016994374914,5.41206908565353E-14));
#138188=DIRECTION('ref_axis',(0.309016994374914,0.951056516295164,6.82961998416067E-15));
#138189=DIRECTION('center_axis',(-0.951056516295158,0.309016994374935,2.02392930158878E-15));
#138190=DIRECTION('ref_axis',(0.309016994374935,0.951056516295158,6.82961998416066E-15));
#138191=DIRECTION('center_axis',(0.951056516295165,-0.309016994374914,-2.15785413849081E-15));
#138192=DIRECTION('ref_axis',(-0.309016994374914,-0.951056516295164,-6.82961998416067E-15));
#138193=DIRECTION('center_axis',(-0.503987876168997,0.163755587629873,0.848045003637578));
#138194=DIRECTION('ref_axis',(-0.859649462041482,-4.46729327993359E-16,
-0.510884333691874));
#138195=DIRECTION('center_axis',(0.475533164204451,-0.154510091261954,-0.86602242548327));
#138196=DIRECTION('ref_axis',(0.876548714628815,-1.69396669624288E-15,0.481313152617475));
#138197=DIRECTION('center_axis',(0.503987855975045,-0.163755558324557,-0.848045021297508));
#138198=DIRECTION('ref_axis',(0.807862963765421,-0.257959309137511,0.529919264233192));
#138199=DIRECTION('center_axis',(-0.503987822791223,0.163755570286383,0.848045038708643));
#138200=DIRECTION('ref_axis',(-0.859649495083693,8.62473446481745E-16,-0.510884278092752));
#138201=DIRECTION('center_axis',(0.475533180627887,-0.154510085541456,-0.86602241748577));
#138202=DIRECTION('ref_axis',(0.825033325009512,-0.26328693971363,0.49999999999998));
#138203=DIRECTION('center_axis',(0.823639804208726,-0.267653025932087,-0.499979330205169));
#138204=DIRECTION('ref_axis',(0.475210466543723,-0.155418826433036,0.866036951219447));
#138205=DIRECTION('center_axis',(0.308786358060973,0.951131423661021,-1.9341749481394E-14));
#138206=DIRECTION('ref_axis',(0.951131423661021,-0.308786358060973,-3.41480999208049E-15));
#138207=DIRECTION('center_axis',(-0.951056516295158,0.309016994374935,2.02392930158878E-15));
#138208=DIRECTION('ref_axis',(0.309016994374935,0.951056516295158,6.82961998416066E-15));
#138209=DIRECTION('center_axis',(0.951056516295165,-0.309016994374914,-2.15785413849081E-15));
#138210=DIRECTION('ref_axis',(-0.309016994374914,-0.951056516295164,-6.82961998416067E-15));
#138211=DIRECTION('center_axis',(-6.89206998773264E-18,-7.02647749501056E-15,
1.));
#138212=DIRECTION('ref_axis',(0.,-1.,-7.02379957427519E-15));
#138213=DIRECTION('center_axis',(0.309247612517378,0.95098155300316,6.64066869178919E-15));
#138214=DIRECTION('ref_axis',(0.95098155300316,-0.309247612517378,-3.41480999208029E-15));
#138215=DIRECTION('center_axis',(0.503988317040571,-0.163755730877738,0.848044713969323));
#138216=DIRECTION('ref_axis',(-0.859649189130473,-2.30534688053848E-17,
0.510884792910614));
#138217=DIRECTION('center_axis',(0.503987822791218,-0.163755570286381,-0.848045038708647));
#138218=DIRECTION('ref_axis',(0.859649495083696,-1.39187210333192E-15,0.510884278092747));
#138219=DIRECTION('center_axis',(0.503988340265106,-0.163755764942529,0.848044693589265));
#138220=DIRECTION('ref_axis',(-0.807930997365388,0.257746148158916,0.529919264233158));
#138221=DIRECTION('center_axis',(0.503988379172015,-0.163755751065492,0.848044673146729));
#138222=DIRECTION('ref_axis',(-0.859649150669458,1.48905909758926E-15,0.510884857627704));
#138223=DIRECTION('center_axis',(-0.503987856145286,0.163755558312952,0.848045021198575));
#138224=DIRECTION('ref_axis',(0.805199544412657,-0.266156471032046,0.529919264233163));
#138225=DIRECTION('center_axis',(0.503987876168979,-0.163755587629867,-0.84804500363759));
#138226=DIRECTION('ref_axis',(0.859649462041493,-6.96683555657854E-16,0.510884333691856));
#138227=DIRECTION('center_axis',(0.308771440182783,0.951136266645033,1.57550132814483E-14));
#138228=DIRECTION('ref_axis',(0.951136266645033,-0.308771440182783,-3.41480999208041E-15));
#138229=DIRECTION('center_axis',(0.951056516295165,-0.309016994374914,-1.05997286994034E-14));
#138230=DIRECTION('ref_axis',(-0.309016994374914,-0.951056516295164,-6.82961998416067E-15));
#138231=DIRECTION('center_axis',(-6.89206998773264E-18,-7.02647749501056E-15,
1.));
#138232=DIRECTION('ref_axis',(0.,-1.,-7.02668578204321E-15));
#138233=DIRECTION('center_axis',(0.309262527968943,0.95097670255073,6.6406348212609E-15));
#138234=DIRECTION('ref_axis',(0.950976702550729,-0.309262527968943,-3.4148099920803E-15));
#138235=DIRECTION('center_axis',(0.951056516295158,-0.309016994374935,-2.02392930158878E-15));
#138236=DIRECTION('ref_axis',(-0.309016994374935,-0.951056516295158,-6.82961998416063E-15));
#138237=DIRECTION('center_axis',(0.823641557783743,-0.267585776504145,0.50001243634958));
#138238=DIRECTION('ref_axis',(0.475234043086884,-0.155453534505877,-0.866017784402216));
#138239=DIRECTION('center_axis',(-0.503988379172015,0.163755751065439,-0.848044673146739));
#138240=DIRECTION('ref_axis',(0.859649150669461,-1.39074635011745E-15,-0.510884857627699));
#138241=DIRECTION('center_axis',(-0.475533019435549,0.154510054854217,-0.86602251147153));
#138242=DIRECTION('ref_axis',(-0.822244813613241,0.271870311888071,0.50000000000001));
#138243=DIRECTION('center_axis',(0.475533035318005,-0.154510049384226,0.866022503726392));
#138244=DIRECTION('ref_axis',(-0.876548788012513,1.21600309223843E-16,0.481313018973926));
#138245=DIRECTION('center_axis',(-0.503988340058923,0.163755764948669,-0.848044693710613));
#138246=DIRECTION('ref_axis',(-0.805129291876817,0.266368911017192,0.529919264233195));
#138247=DIRECTION('center_axis',(-0.503988317040557,0.163755730877758,-0.848044713969328));
#138248=DIRECTION('ref_axis',(0.85964918913048,-5.66681152953988E-16,-0.510884792910601));
#138249=DIRECTION('center_axis',(0.951056516295165,-0.309016994374914,5.82468571404663E-14));
#138250=DIRECTION('ref_axis',(-0.309016994374914,-0.951056516295164,-6.82961998416066E-15));
#138251=DIRECTION('center_axis',(-0.951056516295165,0.309016994374914,2.15785413849081E-15));
#138252=DIRECTION('ref_axis',(0.309016994374914,0.951056516295164,6.82961998416067E-15));
#138253=DIRECTION('center_axis',(0.951056516295158,-0.309016994374935,-2.02392930158878E-15));
#138254=DIRECTION('ref_axis',(-0.309016994374935,-0.951056516295158,-6.82961998416063E-15));
#138255=DIRECTION('center_axis',(0.951056516295165,-0.309016994374914,4.13631080186411E-14));
#138256=DIRECTION('ref_axis',(-0.309016994374914,-0.951056516295164,-6.82961998416067E-15));
#138257=DIRECTION('center_axis',(0.951056516295158,-0.309016994374935,-2.02392930158878E-15));
#138258=DIRECTION('ref_axis',(-0.309016994374935,-0.951056516295158,-6.82961998416063E-15));
#138259=DIRECTION('center_axis',(-0.823661100222748,0.267587483540072,0.499979330205304));
#138260=DIRECTION('ref_axis',(0.475806237447156,-0.153585232132039,0.866036951219362));
#138261=DIRECTION('center_axis',(0.475533164204429,-0.154510091261951,-0.866022425483282));
#138262=DIRECTION('ref_axis',(0.876548714628827,1.19088306137351E-15,0.481313152617452));
#138263=DIRECTION('center_axis',(0.475533172742175,-0.154510094036062,-0.866022420300265));
#138264=DIRECTION('ref_axis',(0.309016994373383,0.951056516295662,-9.35384750808893E-13));
#138265=DIRECTION('center_axis',(-0.489078705150942,0.103956887952922,-0.866022508723083));
#138266=DIRECTION('ref_axis',(-0.207911690818889,-0.978147600733565,6.4690160639327E-13));
#138267=DIRECTION('center_axis',(-0.847087400906983,0.18008469874679,-0.500012436347268));
#138268=DIRECTION('ref_axis',(0.489291521289685,-0.102990311634942,-0.866017784403625));
#138269=DIRECTION('center_axis',(0.489078713616366,-0.103956889752297,0.866022503726312));
#138270=DIRECTION('ref_axis',(-0.870740345484705,1.09228964843654E-16,0.491743073916834));
#138271=DIRECTION('center_axis',(0.978147600733806,-0.207911690817757,-1.45183957723504E-15));
#138272=DIRECTION('ref_axis',(-0.207911690817757,-0.978147600733806,-6.8296199841607E-15));
#138273=DIRECTION('center_axis',(-0.978147600733808,0.207911690817747,1.31409985761785E-15));
#138274=DIRECTION('ref_axis',(0.207911690817747,0.978147600733808,6.82961998416066E-15));
#138275=DIRECTION('center_axis',(-0.978147600733807,0.207911690817754,4.29175525433411E-15));
#138276=DIRECTION('ref_axis',(0.207911690817754,0.978147600733807,6.82961998416071E-15));
#138277=DIRECTION('center_axis',(-0.978147600733808,0.207911690817747,1.31409985761785E-15));
#138278=DIRECTION('ref_axis',(0.207911690817747,0.978147600733808,6.82961998416066E-15));
#138279=DIRECTION('center_axis',(0.978147600733806,-0.207911690817757,-1.45183957723504E-15));
#138280=DIRECTION('ref_axis',(-0.207911690817757,-0.978147600733806,-6.8296199841607E-15));
#138281=DIRECTION('center_axis',(-0.518344097776651,0.110177439185346,0.848045003637584));
#138282=DIRECTION('ref_axis',(-0.85323958281187,-1.42754706638066E-15,-0.521519140898036));
#138283=DIRECTION('center_axis',(0.489078846174035,-0.103956917928307,-0.866022425483268));
#138284=DIRECTION('ref_axis',(0.870740269393757,1.01377976619987E-15,0.491743208652735));
#138285=DIRECTION('center_axis',(0.518344074629046,-0.110177412156386,-0.848045021297502));
#138286=DIRECTION('ref_axis',(0.830401496087484,-0.172101506937531,0.529919264233242));
#138287=DIRECTION('center_axis',(-0.518344042878405,0.110177427516364,0.848045038708645));
#138288=DIRECTION('ref_axis',(-0.853239616987299,-8.10318245671903E-16,
-0.521519084984784));
#138289=DIRECTION('center_axis',(0.489078861909158,-0.103956910524381,-0.866022417485753));
#138290=DIRECTION('ref_axis',(0.848034685338132,-0.175605160697131,0.49999999999999));
#138291=DIRECTION('center_axis',(0.847105178672072,-0.180092991630959,-0.499979330205128));
#138292=DIRECTION('ref_axis',(0.488852904976457,-0.104894406040358,0.866036951219473));
#138293=DIRECTION('center_axis',(0.207674488001815,0.978197989689809,6.83072005339167E-15));
#138294=DIRECTION('ref_axis',(0.978197989689809,-0.207674488001815,-2.10582014878174E-29));
#138295=DIRECTION('center_axis',(-0.978147600733808,0.207911690817747,1.31409985761785E-15));
#138296=DIRECTION('ref_axis',(0.207911690817747,0.978147600733808,6.82961998416066E-15));
#138297=DIRECTION('center_axis',(0.978147600733806,-0.207911690817757,-1.45183957723504E-15));
#138298=DIRECTION('ref_axis',(-0.207911690817757,-0.978147600733806,-6.8296199841607E-15));
#138299=DIRECTION('center_axis',(-3.07718727278846E-18,-7.01224015889347E-15,
1.));
#138300=DIRECTION('ref_axis',(0.,-1.,-7.00969555906581E-15));
#138301=DIRECTION('center_axis',(0.208148881407602,0.978097154258596,6.83001592333892E-15));
#138302=DIRECTION('ref_axis',(0.978097154258596,-0.208148881407602,-3.24411496833464E-30));
#138303=DIRECTION('center_axis',(0.518344551206563,-0.110177535564874,0.848044713969327));
#138304=DIRECTION('ref_axis',(-0.853239300541052,-1.56430135117269E-15,
0.521519602711361));
#138305=DIRECTION('center_axis',(0.51834404287839,-0.11017742751636,-0.848045038708654));
#138306=DIRECTION('ref_axis',(0.853239616987309,1.0828167418591E-16,0.521519084984769));
#138307=DIRECTION('center_axis',(0.518344577866913,-0.110177567004444,0.84804469358929));
#138308=DIRECTION('ref_axis',(-0.830446875604022,0.171882402223312,0.529919264233206));
#138309=DIRECTION('center_axis',(0.518344615107839,-0.110177549147496,0.848044673146738));
#138310=DIRECTION('ref_axis',(-0.853239260760972,-1.65434113834715E-15,
0.521519667794101));
#138311=DIRECTION('center_axis',(-0.518344074799165,0.110177412117555,0.848045021198566));
#138312=DIRECTION('ref_axis',(0.828609503962607,-0.180532167043603,0.529919264233131));
#138313=DIRECTION('center_axis',(0.518344097776644,-0.110177439185345,-0.848045003637588));
#138314=DIRECTION('ref_axis',(0.853239582811875,1.17437859349562E-15,0.521519140898029));
#138315=DIRECTION('center_axis',(0.207659145615641,0.978201246800566,6.83074279767453E-15));
#138316=DIRECTION('ref_axis',(0.978201246800566,-0.207659145615641,-3.71317093631252E-29));
#138317=DIRECTION('center_axis',(0.978147600733807,-0.207911690817754,-1.45183957723502E-15));
#138318=DIRECTION('ref_axis',(-0.207911690817754,-0.978147600733807,-6.8296199841607E-15));
#138319=DIRECTION('center_axis',(-3.07718727278846E-18,-7.01224015889347E-15,
1.));
#138320=DIRECTION('ref_axis',(0.,-1.,-7.01167149618415E-15));
#138321=DIRECTION('center_axis',(0.208164222161082,0.978093889466687,-4.54346712784961E-15));
#138322=DIRECTION('ref_axis',(0.978093889466687,-0.208164222161082,-1.72376173614108E-29));
#138323=DIRECTION('center_axis',(0.978147600733808,-0.207911690817747,-1.31409985761785E-15));
#138324=DIRECTION('ref_axis',(-0.207911690817747,-0.978147600733808,-6.82961998416061E-15));
#138325=DIRECTION('center_axis',(0.847099893161665,-0.180025927305153,0.500012436348753));
#138326=DIRECTION('ref_axis',(0.48887998035015,-0.104926459537374,-0.866017784402716));
#138327=DIRECTION('center_axis',(-0.518344615107841,0.110177549147469,-0.84804467314674));
#138328=DIRECTION('ref_axis',(0.853239260760972,1.65387964661466E-15,-0.521519667794101));
#138329=DIRECTION('center_axis',(-0.489078698392291,0.103956896853528,-0.866022511471548));
#138330=DIRECTION('ref_axis',(-0.846158656401361,0.18443299107549,0.499999999999992));
#138331=DIRECTION('center_axis',(0.489078713616248,-0.103956889752271,0.866022503726381));
#138332=DIRECTION('ref_axis',(-0.870740345484772,7.4899534609633E-16,0.491743073916715));
#138333=DIRECTION('center_axis',(-0.518344577661002,0.110177567039477,-0.848044693710596));
#138334=DIRECTION('ref_axis',(-0.828561842309103,0.180750786620236,0.529919264233252));
#138335=DIRECTION('center_axis',(-0.518344551206586,0.11017753556482,-0.84804471396932));
#138336=DIRECTION('ref_axis',(0.85323930054104,-8.46008946842943E-16,-0.521519602711381));
#138337=DIRECTION('center_axis',(0.978147600733807,-0.207911690817754,-1.45183957723502E-15));
#138338=DIRECTION('ref_axis',(-0.207911690817754,-0.978147600733807,-6.8296199841607E-15));
#138339=DIRECTION('center_axis',(-0.978147600733807,0.207911690817754,1.45183957723502E-15));
#138340=DIRECTION('ref_axis',(0.207911690817754,0.978147600733807,6.8296199841607E-15));
#138341=DIRECTION('center_axis',(0.978147600733808,-0.207911690817747,-1.31409985761785E-15));
#138342=DIRECTION('ref_axis',(-0.207911690817747,-0.978147600733808,-6.82961998416061E-15));
#138343=DIRECTION('center_axis',(0.978147600733807,-0.207911690817754,-5.48948507886774E-14));
#138344=DIRECTION('ref_axis',(-0.207911690817754,-0.978147600733807,-6.82961998416085E-15));
#138345=DIRECTION('center_axis',(0.978147600733808,-0.207911690817747,-1.31409985761785E-15));
#138346=DIRECTION('ref_axis',(-0.207911690817747,-0.978147600733808,-6.82961998416061E-15));
#138347=DIRECTION('center_axis',(-0.847119506978909,0.180025582247284,0.499979330205096));
#138348=DIRECTION('ref_axis',(0.489253749388308,-0.103008581350974,0.866036951219486));
#138349=DIRECTION('center_axis',(0.489078846174003,-0.103956917928279,-0.866022425483289));
#138350=DIRECTION('ref_axis',(0.870740269393776,1.33909771088141E-16,0.491743208652702));
#138351=DIRECTION('center_axis',(0.489078854947432,-0.103956919793121,-0.866022420304715));
#138352=DIRECTION('ref_axis',(0.207911690812507,0.978147600734922,-3.08152452956608E-12));
#138353=DIRECTION('center_axis',(-0.497265934578267,0.0522647557775134,
-0.86602250872106));
#138354=DIRECTION('ref_axis',(-0.104528463268336,-0.994521895368201,3.84644198399901E-13));
#138355=DIRECTION('center_axis',(-0.861270944310119,0.0905534316538301,
-0.500012436348208));
#138356=DIRECTION('ref_axis',(0.497376550147982,-0.0512812291239624,-0.866017784403084));
#138357=DIRECTION('center_axis',(0.497265943181925,-0.0522647566817473,
0.866022503726311));
#138358=DIRECTION('ref_axis',(-0.867207748104374,-6.20026837782905E-15,
0.497946504785143));
#138359=DIRECTION('center_axis',(0.994521895368276,-0.104528463267629,-7.29918357753754E-16));
#138360=DIRECTION('ref_axis',(-0.104528463267629,-0.994521895368276,-6.82961998416064E-15));
#138361=DIRECTION('center_axis',(-0.994521895368275,0.10452846326764,5.89872860613779E-16));
#138362=DIRECTION('ref_axis',(0.10452846326764,0.994521895368275,6.82961998416066E-15));
#138363=DIRECTION('center_axis',(-0.994521895368276,0.104528463267629,7.29918357753754E-16));
#138364=DIRECTION('ref_axis',(0.104528463267629,0.994521895368276,6.82961998416064E-15));
#138365=DIRECTION('center_axis',(-0.994521895368275,0.10452846326764,5.89872860613779E-16));
#138366=DIRECTION('ref_axis',(0.10452846326764,0.994521895368275,6.82961998416066E-15));
#138367=DIRECTION('center_axis',(0.994521895368276,-0.10452846326763,-7.29918357753759E-16));
#138368=DIRECTION('ref_axis',(-0.10452846326763,-0.994521895368276,-6.82961998416064E-15));
#138369=DIRECTION('center_axis',(-0.527021232978627,0.0553921636609735,
0.848045003637569));
#138370=DIRECTION('ref_axis',(-0.849349030019368,7.51365298055634E-15,-0.527831625809934));
#138371=DIRECTION('center_axis',(0.497266077958573,-0.0522647708473797,
-0.866022425483295));
#138372=DIRECTION('ref_axis',(0.867207670398082,-6.90944293724234E-15,0.497946640115919));
#138373=DIRECTION('center_axis',(0.527021207133031,-0.0553921391946541,
-0.848045021297503));
#138374=DIRECTION('ref_axis',(0.843841975853669,-0.0843581245756499,0.529919264233199));
#138375=DIRECTION('center_axis',(-0.527021177161347,0.055392157794341,0.84804503870865));
#138376=DIRECTION('ref_axis',(-0.849349064867519,7.13597841401006E-15,-0.527831569734769));
#138377=DIRECTION('center_axis',(0.497266092833649,-0.0522647618388216,
-0.866022417485765));
#138378=DIRECTION('ref_axis',(0.861744800189553,-0.0859994148019896,0.499999999999982));
#138379=DIRECTION('center_axis',(0.861289491529666,-0.0905598208266563,
-0.499979330205173));
#138380=DIRECTION('ref_axis',(0.497139368682358,-0.0532207405870175,0.866036951219448));
#138381=DIRECTION('center_axis',(0.104287292793425,0.994547213842469,6.94488607545883E-15));
#138382=DIRECTION('ref_axis',(0.994547213842469,-0.104287292793425,-7.04137303703978E-30));
#138383=DIRECTION('center_axis',(-0.994521895368275,0.10452846326764,5.89872860613779E-16));
#138384=DIRECTION('ref_axis',(0.10452846326764,0.994521895368275,6.82961998416066E-15));
#138385=DIRECTION('center_axis',(0.994521895368276,-0.10452846326763,-7.29918357753759E-16));
#138386=DIRECTION('ref_axis',(-0.10452846326763,-0.994521895368276,-6.82961998416064E-15));
#138387=DIRECTION('center_axis',(-7.71409749858844E-19,-6.99768205256557E-15,
1.));
#138388=DIRECTION('ref_axis',(0.,-1.,-6.99559154385642E-15));
#138389=DIRECTION('center_axis',(0.104769627595152,0.994496518411992,6.94453207115987E-15));
#138390=DIRECTION('ref_axis',(0.994496518411992,-0.104769627595152,-1.55544708777506E-29));
#138391=DIRECTION('center_axis',(0.527021693999021,-0.0553922121161813,
0.848044713969304));
#138392=DIRECTION('ref_axis',(-0.849348742192388,-6.71201041252531E-15,
0.527832088960314));
#138393=DIRECTION('center_axis',(0.527021177161445,-0.0553921577943047,
-0.848045038708591));
#138394=DIRECTION('ref_axis',(0.849349064867459,-7.06533916556894E-15,0.527831569734866));
#138395=DIRECTION('center_axis',(0.527021723799459,-0.0553922405982832,
0.848044693589288));
#138396=DIRECTION('ref_axis',(-0.843864204095891,0.084135476703687,0.529919264233196));
#138397=DIRECTION('center_axis',(0.527021758969976,-0.0553922189449034,
0.848044673146735));
#138398=DIRECTION('ref_axis',(-0.849348701629309,-6.7822964013418E-15,0.527832154231445));
#138399=DIRECTION('center_axis',(-0.52702120729681,0.0553921391509293,0.848045021198578));
#138400=DIRECTION('ref_axis',(0.842941044393908,-0.0929299148319318,0.529919264233183));
#138401=DIRECTION('center_axis',(0.527021232978636,-0.0553921636609745,
-0.848045003637563));
#138402=DIRECTION('ref_axis',(0.849349030019363,-7.39781141104914E-15,0.527831625809943));
#138403=DIRECTION('center_axis',(0.10427169399366,0.994548849394384,1.94343765541562E-14));
#138404=DIRECTION('ref_axis',(0.994548849394384,-0.10427169399366,1.05093255583232E-28));
#138405=DIRECTION('center_axis',(0.994521895368276,-0.104528463267629,-7.29918357753754E-16));
#138406=DIRECTION('ref_axis',(-0.104528463267629,-0.994521895368276,-6.82961998416064E-15));
#138407=DIRECTION('center_axis',(-7.71409749858844E-19,-6.99768205256557E-15,
1.));
#138408=DIRECTION('ref_axis',(0.,-1.,-6.99665721032508E-15));
#138409=DIRECTION('center_axis',(0.104785225574074,0.99449487505034,6.94452059562679E-15));
#138410=DIRECTION('ref_axis',(0.994494875050339,-0.104785225574074,2.30312721721348E-29));
#138411=DIRECTION('center_axis',(0.994521895368275,-0.10452846326764,-5.89872860613779E-16));
#138412=DIRECTION('ref_axis',(-0.10452846326764,-0.994521895368275,-6.82961998416068E-15));
#138413=DIRECTION('center_axis',(0.861277224843014,-0.0904936763731455,
0.500012436348527));
#138414=DIRECTION('ref_axis',(0.49716964624011,-0.0532497883133837,-0.866017784402875));
#138415=DIRECTION('center_axis',(-0.527021758969983,0.0553922189449046,
-0.84804467314673));
#138416=DIRECTION('ref_axis',(0.849348701629304,6.78821573216834E-15,-0.527832154231452));
#138417=DIRECTION('center_axis',(-0.497265928783043,0.0522647653398099,
-0.866022511471563));
#138418=DIRECTION('ref_axis',(-0.86080180787837,0.0949749838292013,0.499999999999973));
#138419=DIRECTION('center_axis',(0.497265943181779,-0.0522647566817799,
0.866022503726393));
#138420=DIRECTION('ref_axis',(-0.867207748104458,-6.7740073172956E-15,0.497946504784997));
#138421=DIRECTION('center_axis',(-0.527021723597956,0.0553922406580129,
-0.848044693710611));
#138422=DIRECTION('ref_axis',(-0.842916495801727,0.0931523188110504,0.529919264233205));
#138423=DIRECTION('center_axis',(-0.527021693999002,0.0553922121161323,
-0.848044713969319));
#138424=DIRECTION('ref_axis',(0.849348742192401,6.32826558914321E-15,-0.527832088960293));
#138425=DIRECTION('center_axis',(0.994521895368276,-0.104528463267629,-2.15769772104614E-15));
#138426=DIRECTION('ref_axis',(-0.104528463267629,-0.994521895368276,-6.82961998416064E-15));
#138427=DIRECTION('center_axis',(-0.994521895368276,0.104528463267628,7.29918357753744E-16));
#138428=DIRECTION('ref_axis',(0.104528463267628,0.994521895368276,6.82961998416064E-15));
#138429=DIRECTION('center_axis',(0.994521895368275,-0.10452846326764,-5.89872860613779E-16));
#138430=DIRECTION('ref_axis',(-0.10452846326764,-0.994521895368275,-6.82961998416068E-15));
#138431=DIRECTION('center_axis',(0.994521895368276,-0.104528463267629,-1.60286761075628E-17));
#138432=DIRECTION('ref_axis',(-0.104528463267629,-0.994521895368276,-6.82961998416064E-15));
#138433=DIRECTION('center_axis',(0.994521895368275,-0.10452846326764,-5.89872860613779E-16));
#138434=DIRECTION('ref_axis',(-0.10452846326764,-0.994521895368275,-6.82961998416068E-15));
#138435=DIRECTION('center_axis',(-0.861296695145334,0.0904912830026632,
0.499979330205017));
#138436=DIRECTION('ref_axis',(0.497340894868541,-0.0513033470031167,0.86603695121954));
#138437=DIRECTION('center_axis',(0.497266077958562,-0.0522647708473785,
-0.866022425483302));
#138438=DIRECTION('ref_axis',(0.867207670398088,-6.98667298451095E-15,0.497946640115907));
#138439=DIRECTION('center_axis',(0.49726608688627,-0.0522647717857253,-0.866022420300423));
#138440=DIRECTION('ref_axis',(0.104528463273401,0.994521895367669,3.35252384984286E-12));
#138441=DIRECTION('center_axis',(0.,0.,1.));
#138442=DIRECTION('ref_axis',(1.,0.,0.));
#138443=DIRECTION('center_axis',(0.,0.,1.));
#138444=DIRECTION('ref_axis',(1.,0.,0.));
#138445=DIRECTION('center_axis',(1.22464679914735E-16,-1.,0.));
#138446=DIRECTION('ref_axis',(-1.,-1.22464679914735E-16,0.));
#138447=DIRECTION('center_axis',(0.,0.,-1.));
#138448=DIRECTION('ref_axis',(1.,0.,0.));
#138449=DIRECTION('center_axis',(0.,0.,1.));
#138450=DIRECTION('ref_axis',(1.,0.,0.));
#138451=DIRECTION('center_axis',(0.,0.,1.));
#138452=DIRECTION('ref_axis',(1.,0.,0.));
#138453=DIRECTION('center_axis',(-1.22464679914735E-16,1.,0.));
#138454=DIRECTION('ref_axis',(-1.,-1.22464679914735E-16,0.));
#138455=DIRECTION('center_axis',(0.,0.,-1.));
#138456=DIRECTION('ref_axis',(1.,0.,0.));
#138457=DIRECTION('center_axis',(0.,0.,-1.));
#138458=DIRECTION('ref_axis',(-1.,0.,0.));
#138459=DIRECTION('center_axis',(0.,0.,-1.));
#138460=DIRECTION('ref_axis',(-1.,0.,0.));
#138461=DIRECTION('center_axis',(-1.22464679914735E-16,-1.,0.));
#138462=DIRECTION('ref_axis',(1.,-1.22464679914735E-16,0.));
#138463=DIRECTION('center_axis',(0.,0.,1.));
#138464=DIRECTION('ref_axis',(-1.,0.,0.));
#138465=DIRECTION('center_axis',(0.,0.,1.));
#138466=DIRECTION('ref_axis',(-1.,0.,0.));
#138467=DIRECTION('center_axis',(0.,0.,1.));
#138468=DIRECTION('ref_axis',(1.,0.,0.));
#138469=DIRECTION('center_axis',(0.,0.,1.));
#138470=DIRECTION('ref_axis',(1.,0.,0.));
#138471=DIRECTION('',(0.,0.,1.));
#138472=DIRECTION('center_axis',(0.,0.,1.));
#138473=DIRECTION('ref_axis',(1.,0.,0.));
#138474=DIRECTION('',(0.,0.,1.));
#138475=DIRECTION('center_axis',(0.,0.,1.));
#138476=DIRECTION('ref_axis',(1.,0.,0.));
#138477=DIRECTION('center_axis',(0.,0.,-1.));
#138478=DIRECTION('ref_axis',(-1.,0.,0.));
#138479=DIRECTION('',(0.,0.,-1.));
#138480=DIRECTION('center_axis',(0.,0.,-1.));
#138481=DIRECTION('ref_axis',(-1.,0.,0.));
#138482=DIRECTION('center_axis',(0.,0.,-1.));
#138483=DIRECTION('ref_axis',(-1.,0.,0.));
#138484=DIRECTION('center_axis',(0.,0.,-1.));
#138485=DIRECTION('ref_axis',(-1.,0.,0.));
#138486=DIRECTION('center_axis',(0.,0.,1.));
#138487=DIRECTION('ref_axis',(1.,0.,0.));
#138488=DIRECTION('center_axis',(0.,0.,1.));
#138489=DIRECTION('ref_axis',(1.,0.,0.));
#138490=DIRECTION('center_axis',(0.,0.,1.));
#138491=DIRECTION('ref_axis',(1.,0.,0.));
#138492=DIRECTION('center_axis',(1.22464679914735E-16,-1.,0.));
#138493=DIRECTION('ref_axis',(-1.,-1.22464679914735E-16,0.));
#138494=DIRECTION('center_axis',(0.,0.,-1.));
#138495=DIRECTION('ref_axis',(1.,0.,0.));
#138496=DIRECTION('center_axis',(0.,0.,1.));
#138497=DIRECTION('ref_axis',(1.,0.,0.));
#138498=DIRECTION('center_axis',(0.,0.,1.));
#138499=DIRECTION('ref_axis',(1.,0.,0.));
#138500=DIRECTION('center_axis',(1.22464679914735E-16,-1.,0.));
#138501=DIRECTION('ref_axis',(-1.,-1.22464679914735E-16,0.));
#138502=DIRECTION('center_axis',(0.,0.,-1.));
#138503=DIRECTION('ref_axis',(1.,0.,0.));
#138504=DIRECTION('center_axis',(0.,0.,1.));
#138505=DIRECTION('ref_axis',(1.,0.,0.));
#138506=DIRECTION('center_axis',(0.,0.,1.));
#138507=DIRECTION('ref_axis',(1.,0.,0.));
#138508=DIRECTION('',(0.,0.,1.));
#138509=DIRECTION('center_axis',(0.,0.,1.));
#138510=DIRECTION('ref_axis',(1.,0.,0.));
#138511=DIRECTION('',(0.,0.,-1.));
#138512=DIRECTION('center_axis',(0.,0.,1.));
#138513=DIRECTION('ref_axis',(1.,0.,0.));
#138514=DIRECTION('center_axis',(0.,0.,1.));
#138515=DIRECTION('ref_axis',(1.,0.,0.));
#138516=DIRECTION('center_axis',(0.,0.,1.));
#138517=DIRECTION('ref_axis',(1.,0.,0.));
#138518=DIRECTION('center_axis',(0.,0.,1.));
#138519=DIRECTION('ref_axis',(1.,0.,0.));
#138520=DIRECTION('center_axis',(0.,0.,-1.));
#138521=DIRECTION('ref_axis',(1.,0.,0.));
#138522=DIRECTION('center_axis',(1.22464679914735E-16,-1.,0.));
#138523=DIRECTION('ref_axis',(-1.,-1.22464679914735E-16,0.));
#138524=DIRECTION('center_axis',(0.,0.,-1.));
#138525=DIRECTION('ref_axis',(1.,0.,0.));
#138526=DIRECTION('center_axis',(0.,0.,1.));
#138527=DIRECTION('ref_axis',(-1.83697019872103E-16,-1.,0.));
#138528=DIRECTION('center_axis',(0.,0.,-1.));
#138529=DIRECTION('ref_axis',(-1.,0.,0.));
#138530=DIRECTION('center_axis',(-0.990048018535926,0.14072995769589,0.));
#138531=DIRECTION('ref_axis',(-0.14072995769589,-0.990048018535926,0.));
#138532=DIRECTION('center_axis',(0.,0.,1.));
#138533=DIRECTION('ref_axis',(1.,0.,0.));
#138534=DIRECTION('center_axis',(-0.990048018535926,-0.140729957695892,
0.));
#138535=DIRECTION('ref_axis',(0.140729957695892,-0.990048018535926,0.));
#138536=DIRECTION('center_axis',(0.,0.,1.));
#138537=DIRECTION('ref_axis',(1.,0.,0.));
#138538=DIRECTION('center_axis',(0.,0.,-1.));
#138539=DIRECTION('ref_axis',(1.,0.,0.));
#138540=DIRECTION('center_axis',(0.573576436351042,-0.819152044288994,-9.00692692729371E-16));
#138541=DIRECTION('ref_axis',(0.819152044288994,0.573576436351042,-6.35202185790921E-32));
#138542=DIRECTION('center_axis',(0.,0.,1.));
#138543=DIRECTION('ref_axis',(1.,0.,0.));
#138544=DIRECTION('center_axis',(-0.819152044288994,0.573576436351042,0.));
#138545=DIRECTION('ref_axis',(-0.573576436351042,-0.819152044288994,0.));
#138546=DIRECTION('center_axis',(0.,0.,1.));
#138547=DIRECTION('ref_axis',(1.,0.,0.));
#138548=DIRECTION('center_axis',(0.,0.,-1.));
#138549=DIRECTION('ref_axis',(1.,0.,0.));
#138550=DIRECTION('center_axis',(0.819152044288994,0.573576436351042,-2.6835009273527E-15));
#138551=DIRECTION('ref_axis',(-0.573576436351042,0.819152044288994,-8.18154877134231E-32));
#138552=DIRECTION('center_axis',(0.,0.,1.));
#138553=DIRECTION('ref_axis',(1.,0.,0.));
#138554=DIRECTION('center_axis',(-0.573576436351042,-0.819152044288994,
0.));
#138555=DIRECTION('ref_axis',(0.819152044288994,-0.573576436351042,0.));
#138556=DIRECTION('center_axis',(0.,0.,1.));
#138557=DIRECTION('ref_axis',(1.,0.,0.));
#138558=DIRECTION('center_axis',(-0.309478661079813,-0.950906387788118,
0.));
#138559=DIRECTION('ref_axis',(0.950906387788118,-0.309478661079813,0.));
#138560=DIRECTION('center_axis',(0.,0.,-1.));
#138561=DIRECTION('ref_axis',(1.,-4.09777199049639E-15,0.));
#138562=DIRECTION('center_axis',(0.573576436351045,-0.819152044288993,0.));
#138563=DIRECTION('ref_axis',(0.819152044288993,0.573576436351045,0.));
#138564=DIRECTION('center_axis',(0.,0.,1.));
#138565=DIRECTION('ref_axis',(1.,0.,0.));
#138566=DIRECTION('center_axis',(0.573576436351045,0.819152044288993,1.49186591246458E-15));
#138567=DIRECTION('ref_axis',(-0.819152044288993,0.573576436351045,-8.00341439460267E-32));
#138568=DIRECTION('center_axis',(0.,0.,-1.));
#138569=DIRECTION('ref_axis',(1.,1.36592399683213E-14,0.));
#138570=DIRECTION('center_axis',(0.309478661079813,-0.950906387788118,0.));
#138571=DIRECTION('ref_axis',(0.950906387788118,0.309478661079813,0.));
#138572=DIRECTION('center_axis',(0.,0.,1.));
#138573=DIRECTION('ref_axis',(1.,0.,0.));
#138574=DIRECTION('center_axis',(0.309478661079813,0.950906387788118,0.));
#138575=DIRECTION('ref_axis',(-0.950906387788118,0.309478661079813,0.));
#138576=DIRECTION('center_axis',(0.,0.,-1.));
#138577=DIRECTION('ref_axis',(1.,1.0927391974657E-14,0.));
#138578=DIRECTION('center_axis',(-0.573576436351046,0.819152044288992,0.));
#138579=DIRECTION('ref_axis',(-0.819152044288992,-0.573576436351046,0.));
#138580=DIRECTION('center_axis',(0.,0.,1.));
#138581=DIRECTION('ref_axis',(1.,0.,0.));
#138582=DIRECTION('center_axis',(0.,0.,1.));
#138583=DIRECTION('ref_axis',(1.,0.,0.));
#138584=DIRECTION('center_axis',(0.,0.,-1.));
#138585=DIRECTION('ref_axis',(1.,8.88178419700125E-16,0.));
#138586=DIRECTION('center_axis',(-0.309478661079813,0.950906387788118,0.));
#138587=DIRECTION('ref_axis',(-0.950906387788118,-0.309478661079813,0.));
#138588=DIRECTION('center_axis',(0.,0.,1.));
#138589=DIRECTION('ref_axis',(1.,0.,0.));
#138590=DIRECTION('center_axis',(-0.573576436351046,-0.819152044288992,
-1.49186591246457E-15));
#138591=DIRECTION('ref_axis',(0.819152044288992,-0.573576436351046,-5.52212474718673E-32));
#138592=DIRECTION('center_axis',(0.,0.,-1.));
#138593=DIRECTION('ref_axis',(1.,9.56146797782492E-15,0.));
#138594=DIRECTION('center_axis',(0.,0.,1.));
#138595=DIRECTION('ref_axis',(1.,0.,0.));
#138596=DIRECTION('',(0.,0.,-1.));
#138597=DIRECTION('center_axis',(0.,0.,-1.));
#138598=DIRECTION('ref_axis',(-1.,0.,0.));
#138599=DIRECTION('',(0.,0.,1.));
#138600=DIRECTION('center_axis',(0.,0.,1.));
#138601=DIRECTION('ref_axis',(1.,0.,0.));
#138602=DIRECTION('',(0.,0.,-1.));
#138603=DIRECTION('center_axis',(0.,0.,-1.));
#138604=DIRECTION('ref_axis',(-1.,0.,0.));
#138605=DIRECTION('',(0.,0.,1.));
#138606=DIRECTION('center_axis',(0.,0.,-1.));
#138607=DIRECTION('ref_axis',(-1.,0.,0.));
#138608=DIRECTION('center_axis',(0.,0.,1.));
#138609=DIRECTION('ref_axis',(-1.,0.,0.));
#138610=DIRECTION('center_axis',(0.,0.,-1.));
#138611=DIRECTION('ref_axis',(-1.,0.,0.));
#138612=DIRECTION('center_axis',(0.,0.,-1.));
#138613=DIRECTION('ref_axis',(-1.,0.,0.));
#138614=DIRECTION('center_axis',(0.,0.,-1.));
#138615=DIRECTION('ref_axis',(1.,0.,0.));
#138616=DIRECTION('',(0.,0.,-1.));
#138617=DIRECTION('center_axis',(0.,0.,-1.));
#138618=DIRECTION('ref_axis',(-1.,0.,0.));
#138619=DIRECTION('center_axis',(0.,0.,-1.));
#138620=DIRECTION('ref_axis',(-1.,0.,0.));
#138621=DIRECTION('center_axis',(0.,0.,1.));
#138622=DIRECTION('ref_axis',(1.,0.,0.));
#138623=DIRECTION('',(0.,0.,-1.));
#138624=DIRECTION('center_axis',(0.,0.,-1.));
#138625=DIRECTION('ref_axis',(-1.,0.,0.));
#138626=DIRECTION('center_axis',(0.,0.,-1.));
#138627=DIRECTION('ref_axis',(-1.,0.,0.));
#138628=DIRECTION('center_axis',(0.,0.,1.));
#138629=DIRECTION('ref_axis',(1.,0.,0.));
#138630=DIRECTION('',(0.,0.,-1.));
#138631=DIRECTION('center_axis',(0.,0.,-1.));
#138632=DIRECTION('ref_axis',(-1.,0.,0.));
#138633=DIRECTION('center_axis',(0.,0.,-1.));
#138634=DIRECTION('ref_axis',(-1.,0.,0.));
#138635=DIRECTION('center_axis',(0.,0.,1.));
#138636=DIRECTION('ref_axis',(1.,0.,0.));
#138637=DIRECTION('',(0.,0.,-1.));
#138638=DIRECTION('center_axis',(0.,0.,-1.));
#138639=DIRECTION('ref_axis',(-1.,0.,0.));
#138640=DIRECTION('center_axis',(0.,0.,-1.));
#138641=DIRECTION('ref_axis',(-1.,0.,0.));
#138642=DIRECTION('center_axis',(0.,0.,1.));
#138643=DIRECTION('ref_axis',(1.,0.,0.));
#138644=DIRECTION('',(0.,0.,-1.));
#138645=DIRECTION('center_axis',(0.,0.,-1.));
#138646=DIRECTION('ref_axis',(-1.,0.,0.));
#138647=DIRECTION('center_axis',(0.,0.,1.));
#138648=DIRECTION('ref_axis',(1.,0.,0.));
#138649=DIRECTION('',(0.,0.,1.));
#138650=DIRECTION('center_axis',(0.,0.,-1.));
#138651=DIRECTION('ref_axis',(-1.,0.,0.));
#138652=DIRECTION('',(0.,0.,-1.));
#138653=DIRECTION('center_axis',(0.,0.,-1.));
#138654=DIRECTION('ref_axis',(5.0532154980743E-16,-1.,0.));
#138655=DIRECTION('center_axis',(0.,0.,1.));
#138656=DIRECTION('ref_axis',(-1.,6.21724893790088E-15,0.));
#138657=DIRECTION('center_axis',(0.,0.,1.));
#138658=DIRECTION('ref_axis',(1.,0.,0.));
#138659=DIRECTION('center_axis',(0.,0.,1.));
#138660=DIRECTION('ref_axis',(1.,0.,0.));
#138661=DIRECTION('center_axis',(0.,0.,1.));
#138662=DIRECTION('ref_axis',(-1.,0.,0.));
#138663=DIRECTION('center_axis',(0.,0.,1.));
#138664=DIRECTION('ref_axis',(1.,0.,0.));
#138665=DIRECTION('center_axis',(0.,0.,1.));
#138666=DIRECTION('ref_axis',(-1.,4.44089209850063E-15,0.));
#138667=DIRECTION('center_axis',(0.,0.,1.));
#138668=DIRECTION('ref_axis',(1.,0.,0.));
#138669=DIRECTION('center_axis',(0.,0.,1.));
#138670=DIRECTION('ref_axis',(-1.,-5.32907051820075E-15,0.));
#138671=DIRECTION('center_axis',(0.,0.,-1.));
#138672=DIRECTION('ref_axis',(-1.,0.,0.));
#138673=DIRECTION('center_axis',(0.,0.,-1.));
#138674=DIRECTION('ref_axis',(1.,0.,0.));
#138675=DIRECTION('',(0.,0.,1.));
#138676=DIRECTION('center_axis',(0.,0.,1.));
#138677=DIRECTION('ref_axis',(-1.,0.,0.));
#138678=DIRECTION('',(0.,0.,-1.));
#138679=DIRECTION('center_axis',(0.,0.,-1.));
#138680=DIRECTION('ref_axis',(-1.,0.,0.));
#138681=DIRECTION('',(0.,0.,-1.));
#138682=DIRECTION('center_axis',(0.,0.,1.));
#138683=DIRECTION('ref_axis',(1.,0.,0.));
#138684=DIRECTION('',(0.,0.,1.));
#138685=DIRECTION('center_axis',(0.,0.,-1.));
#138686=DIRECTION('ref_axis',(-1.,0.,0.));
#138687=DIRECTION('center_axis',(0.,0.,-1.));
#138688=DIRECTION('ref_axis',(1.,1.11022302462516E-15,0.));
#138689=DIRECTION('',(0.,0.,1.));
#138690=DIRECTION('center_axis',(0.,0.,1.));
#138691=DIRECTION('ref_axis',(1.,0.,0.));
#138692=DIRECTION('',(0.,0.,-1.));
#138693=DIRECTION('center_axis',(0.,0.,-1.));
#138694=DIRECTION('ref_axis',(-1.,0.,0.));
#138695=DIRECTION('',(0.,0.,-1.));
#138696=DIRECTION('center_axis',(0.,0.,1.));
#138697=DIRECTION('ref_axis',(1.,0.,0.));
#138698=DIRECTION('',(0.,0.,1.));
#138699=DIRECTION('center_axis',(0.,1.,0.));
#138700=DIRECTION('ref_axis',(0.,0.,1.));
#138701=DIRECTION('',(0.,0.,-1.));
#138702=DIRECTION('',(-1.,0.,0.));
#138703=DIRECTION('',(-1.,0.,0.));
#138704=DIRECTION('center_axis',(1.,0.,0.));
#138705=DIRECTION('ref_axis',(0.,0.,-1.));
#138706=DIRECTION('',(0.,1.,0.));
#138707=DIRECTION('',(0.,1.,0.));
#138708=DIRECTION('center_axis',(-1.,0.,0.));
#138709=DIRECTION('ref_axis',(0.,0.,1.));
#138710=DIRECTION('',(0.,0.,-1.));
#138711=DIRECTION('',(0.,-1.,0.));
#138712=DIRECTION('',(0.,0.,-1.));
#138713=DIRECTION('',(0.,-1.,0.));
#138714=DIRECTION('center_axis',(0.,0.,-1.));
#138715=DIRECTION('ref_axis',(0.707106781186548,-0.707106781186547,0.));
#138716=DIRECTION('',(0.,0.,1.));
#138717=DIRECTION('',(0.,0.,1.));
#138718=DIRECTION('center_axis',(0.,0.,1.));
#138719=DIRECTION('ref_axis',(1.,0.,0.));
#138720=DIRECTION('center_axis',(0.,0.,-1.));
#138721=DIRECTION('ref_axis',(-1.,0.,0.));
#138722=DIRECTION('center_axis',(0.,0.,1.));
#138723=DIRECTION('ref_axis',(1.,0.,0.));
#138724=DIRECTION('center_axis',(0.,0.,-1.));
#138725=DIRECTION('ref_axis',(0.707106781186547,0.707106781186547,0.));
#138726=DIRECTION('',(0.,0.,1.));
#138727=DIRECTION('',(0.,0.,1.));
#138728=DIRECTION('center_axis',(0.,0.,1.));
#138729=DIRECTION('ref_axis',(1.,0.,0.));
#138730=DIRECTION('center_axis',(0.,0.,-1.));
#138731=DIRECTION('ref_axis',(-1.,0.,0.));
#138732=DIRECTION('',(0.,0.,-1.));
#138733=DIRECTION('center_axis',(0.,0.,1.));
#138734=DIRECTION('ref_axis',(1.,0.,0.));
#138735=DIRECTION('center_axis',(0.,-1.,0.));
#138736=DIRECTION('ref_axis',(0.,0.,-1.));
#138737=DIRECTION('',(1.,0.,0.));
#138738=DIRECTION('',(1.,0.,0.));
#138739=DIRECTION('',(1.,0.,0.));
#138740=DIRECTION('center_axis',(0.,0.,1.));
#138741=DIRECTION('ref_axis',(1.,0.,0.));
#138742=DIRECTION('',(0.,0.,1.));
#138743=DIRECTION('center_axis',(0.,0.,-1.));
#138744=DIRECTION('ref_axis',(-1.,0.,0.));
#138745=DIRECTION('',(0.,0.,1.));
#138746=DIRECTION('center_axis',(0.,0.,-1.));
#138747=DIRECTION('ref_axis',(-1.,0.,0.));
#138748=DIRECTION('center_axis',(1.,0.,0.));
#138749=DIRECTION('ref_axis',(0.,0.,-1.));
#138750=DIRECTION('',(0.,1.,0.));
#138751=DIRECTION('',(0.,0.,1.));
#138752=DIRECTION('',(0.,1.,0.));
#138753=DIRECTION('center_axis',(0.,0.,1.));
#138754=DIRECTION('ref_axis',(1.,0.,0.));
#138755=DIRECTION('center_axis',(0.,0.,-1.));
#138756=DIRECTION('ref_axis',(-1.,0.,0.));
#138757=DIRECTION('',(0.,0.,1.));
#138758=DIRECTION('center_axis',(0.,0.,-1.));
#138759=DIRECTION('ref_axis',(-1.,0.,0.));
#138760=DIRECTION('center_axis',(-1.5419764230905E-16,-1.,0.));
#138761=DIRECTION('ref_axis',(1.,-1.5419764230905E-16,0.));
#138762=DIRECTION('',(1.,-1.5419764230905E-16,0.));
#138763=DIRECTION('',(0.,0.,1.));
#138764=DIRECTION('',(1.,-1.5419764230905E-16,0.));
#138765=DIRECTION('center_axis',(0.,0.,1.));
#138766=DIRECTION('ref_axis',(1.,0.,0.));
#138767=DIRECTION('center_axis',(0.,0.,-1.));
#138768=DIRECTION('ref_axis',(-1.,0.,0.));
#138769=DIRECTION('',(0.,0.,1.));
#138770=DIRECTION('center_axis',(0.,0.,-1.));
#138771=DIRECTION('ref_axis',(-1.,0.,0.));
#138772=DIRECTION('center_axis',(-1.,7.70988211545247E-17,0.));
#138773=DIRECTION('ref_axis',(-7.70988211545247E-17,-1.,0.));
#138774=DIRECTION('',(-7.70988211545248E-17,-1.,0.));
#138775=DIRECTION('',(0.,0.,1.));
#138776=DIRECTION('',(-7.70988211545248E-17,-1.,0.));
#138777=DIRECTION('center_axis',(0.,0.,1.));
#138778=DIRECTION('ref_axis',(1.,0.,0.));
#138779=DIRECTION('center_axis',(0.,0.,-1.));
#138780=DIRECTION('ref_axis',(-1.,0.,0.));
#138781=DIRECTION('',(0.,0.,1.));
#138782=DIRECTION('center_axis',(0.,0.,-1.));
#138783=DIRECTION('ref_axis',(-1.,0.,0.));
#138784=DIRECTION('center_axis',(0.,1.,0.));
#138785=DIRECTION('ref_axis',(0.,0.,1.));
#138786=DIRECTION('',(-1.,0.,0.));
#138787=DIRECTION('',(-1.,0.,0.));
#138788=DIRECTION('center_axis',(0.,0.,1.));
#138789=DIRECTION('ref_axis',(1.,0.,0.));
#138790=DIRECTION('',(0.,1.,0.));
#138791=DIRECTION('center_axis',(0.,0.,1.));
#138792=DIRECTION('ref_axis',(1.,0.,0.));
#138793=DIRECTION('',(0.,-1.,0.));
#138794=DIRECTION('center_axis',(1.,0.,0.));
#138795=DIRECTION('ref_axis',(0.,0.,-1.));
#138796=DIRECTION('',(0.,1.,0.));
#138797=DIRECTION('',(0.,0.,1.));
#138798=DIRECTION('',(0.,0.,1.));
#138799=DIRECTION('center_axis',(1.,3.85138571020619E-14,3.57317646046073E-15));
#138800=DIRECTION('ref_axis',(-3.87079718928684E-14,0.99239999161251,0.123053877011211));
#138801=DIRECTION('center_axis',(1.,0.,0.));
#138802=DIRECTION('ref_axis',(0.,0.,-1.));
#138803=DIRECTION('',(0.,0.,1.));
#138804=DIRECTION('',(0.,-1.,0.));
#138805=DIRECTION('center_axis',(-1.,-3.85138571020628E-14,-3.57317646045933E-15));
#138806=DIRECTION('ref_axis',(-3.8560793292515E-14,0.999999998571857,-5.34442274211441E-5));
#138807=DIRECTION('',(0.,0.,-1.));
#138808=DIRECTION('center_axis',(0.,0.,1.));
#138809=DIRECTION('ref_axis',(1.,0.,0.));
#138810=DIRECTION('center_axis',(0.,0.,-1.));
#138811=DIRECTION('ref_axis',(1.,1.24344978758018E-14,0.));
#138812=DIRECTION('center_axis',(0.,0.,1.));
#138813=DIRECTION('ref_axis',(1.,0.,0.));
#138814=DIRECTION('center_axis',(0.,0.,1.));
#138815=DIRECTION('ref_axis',(1.,0.,0.));
#138816=DIRECTION('',(0.,0.,1.));
#138817=DIRECTION('center_axis',(0.,0.,-1.));
#138818=DIRECTION('ref_axis',(-1.,0.,0.));
#138819=DIRECTION('',(0.,0.,-1.));
#138820=DIRECTION('center_axis',(0.,0.,1.));
#138821=DIRECTION('ref_axis',(1.,0.,0.));
#138822=DIRECTION('',(-1.,0.,0.));
#138823=DIRECTION('center_axis',(0.,0.,1.));
#138824=DIRECTION('ref_axis',(1.,0.,0.));
#138825=DIRECTION('center_axis',(0.,0.,1.));
#138826=DIRECTION('ref_axis',(1.,0.,0.));
#138827=DIRECTION('',(-0.819152044288992,-0.573576436351046,0.));
#138828=DIRECTION('center_axis',(0.,0.,1.));
#138829=DIRECTION('ref_axis',(1.,0.,0.));
#138830=DIRECTION('center_axis',(0.,0.,1.));
#138831=DIRECTION('ref_axis',(1.,0.,0.));
#138832=DIRECTION('',(-1.,0.,0.));
#138833=DIRECTION('',(-0.819152044288992,0.573576436351046,0.));
#138834=DIRECTION('center_axis',(0.,0.,1.));
#138835=DIRECTION('ref_axis',(1.,0.,0.));
#138836=DIRECTION('center_axis',(0.,0.,1.));
#138837=DIRECTION('ref_axis',(1.,0.,0.));
#138838=DIRECTION('center_axis',(0.,0.,1.));
#138839=DIRECTION('ref_axis',(1.,0.,0.));
#138840=DIRECTION('center_axis',(0.,0.,-1.));
#138841=DIRECTION('ref_axis',(-1.,0.,0.));
#138842=DIRECTION('',(0.,0.,-1.));
#138843=DIRECTION('',(0.,0.,1.));
#138844=DIRECTION('center_axis',(0.,0.,1.));
#138845=DIRECTION('ref_axis',(1.,0.,0.));
#138846=DIRECTION('',(0.573576436351045,-0.819152044288992,0.));
#138847=DIRECTION('center_axis',(0.,0.,-1.));
#138848=DIRECTION('ref_axis',(1.,-8.88178419700125E-16,0.));
#138849=DIRECTION('',(-0.819152044288992,0.573576436351046,0.));
#138850=DIRECTION('center_axis',(0.,0.,1.));
#138851=DIRECTION('ref_axis',(1.,0.,0.));
#138852=DIRECTION('center_axis',(0.,0.,1.));
#138853=DIRECTION('ref_axis',(-1.,1.22464679914735E-16,0.));
#138854=DIRECTION('center_axis',(0.,0.,1.));
#138855=DIRECTION('ref_axis',(1.,0.,0.));
#138856=DIRECTION('center_axis',(0.,0.,1.));
#138857=DIRECTION('ref_axis',(1.,0.,0.));
#138858=DIRECTION('',(0.819152044288992,0.573576436351046,0.));
#138859=DIRECTION('center_axis',(0.,0.,-1.));
#138860=DIRECTION('ref_axis',(1.,8.88178419700125E-16,0.));
#138861=DIRECTION('',(-0.573576436351045,-0.819152044288992,0.));
#138862=DIRECTION('center_axis',(0.,0.,1.));
#138863=DIRECTION('ref_axis',(1.,0.,0.));
#138864=DIRECTION('center_axis',(0.,0.,1.));
#138865=DIRECTION('ref_axis',(1.,0.,0.));
#138866=DIRECTION('',(0.,0.,-1.));
#138867=DIRECTION('center_axis',(0.,0.,1.));
#138868=DIRECTION('ref_axis',(1.,0.,0.));
#138869=DIRECTION('',(0.,0.,1.));
#138870=DIRECTION('center_axis',(0.,0.,-1.));
#138871=DIRECTION('ref_axis',(-1.,0.,0.));
#138872=DIRECTION('center_axis',(0.,0.,1.));
#138873=DIRECTION('ref_axis',(1.,0.,0.));
#138874=DIRECTION('',(-0.573576436351046,0.819152044288992,0.));
#138875=DIRECTION('center_axis',(0.,0.,-1.));
#138876=DIRECTION('ref_axis',(1.,0.,0.));
#138877=DIRECTION('',(0.819152044288992,-0.573576436351045,0.));
#138878=DIRECTION('center_axis',(0.,0.,1.));
#138879=DIRECTION('ref_axis',(1.,0.,0.));
#138880=DIRECTION('',(-0.819152044288992,-0.573576436351046,0.));
#138881=DIRECTION('center_axis',(0.,0.,-1.));
#138882=DIRECTION('ref_axis',(1.,-4.44089209850063E-15,0.));
#138883=DIRECTION('',(0.573576436351045,0.819152044288992,0.));
#138884=DIRECTION('center_axis',(-0.573576436351046,0.819152044288992,0.));
#138885=DIRECTION('ref_axis',(-0.819152044288992,-0.573576436351046,0.));
#138886=DIRECTION('',(0.,0.,1.));
#138887=DIRECTION('',(0.819152044288992,0.573576436351046,0.));
#138888=DIRECTION('center_axis',(0.573576436351046,0.819152044288992,0.));
#138889=DIRECTION('ref_axis',(-0.819152044288992,0.573576436351046,0.));
#138890=DIRECTION('',(0.819152044288992,-0.573576436351046,0.));
#138891=DIRECTION('',(0.,0.,-1.));
#138892=DIRECTION('center_axis',(-0.819152044288992,-0.573576436351045,
0.));
#138893=DIRECTION('ref_axis',(0.573576436351045,-0.819152044288992,0.));
#138894=DIRECTION('',(-0.573576436351045,0.819152044288992,0.));
#138895=DIRECTION('',(0.573576436351045,-0.819152044288992,0.));
#138896=DIRECTION('center_axis',(0.,0.,1.));
#138897=DIRECTION('ref_axis',(1.,0.,0.));
#138898=DIRECTION('center_axis',(0.,0.,-1.));
#138899=DIRECTION('ref_axis',(1.,-1.59900175447779E-14,0.));
#138900=DIRECTION('',(0.,-1.,0.));
#138901=DIRECTION('center_axis',(0.,0.,-1.));
#138902=DIRECTION('ref_axis',(1.,0.,0.));
#138903=DIRECTION('',(0.573576436351045,0.819152044288992,0.));
#138904=DIRECTION('center_axis',(0.,0.,-1.));
#138905=DIRECTION('ref_axis',(1.,2.66453525910038E-15,0.));
#138906=DIRECTION('',(-0.573576436351045,0.819152044288992,0.));
#138907=DIRECTION('center_axis',(-0.819152044288992,0.573576436351045,0.));
#138908=DIRECTION('ref_axis',(-0.573576436351045,-0.819152044288992,0.));
#138909=DIRECTION('',(0.573576436351045,0.819152044288992,0.));
#138910=DIRECTION('',(-0.573576436351045,-0.819152044288992,0.));
#138911=DIRECTION('center_axis',(0.573576436351046,-0.819152044288992,0.));
#138912=DIRECTION('ref_axis',(0.819152044288992,0.573576436351046,0.));
#138913=DIRECTION('',(0.,0.,1.));
#138914=DIRECTION('',(-0.819152044288992,-0.573576436351046,0.));
#138915=DIRECTION('',(0.819152044288992,0.573576436351046,0.));
#138916=DIRECTION('center_axis',(0.,0.,1.));
#138917=DIRECTION('ref_axis',(1.,0.,0.));
#138918=DIRECTION('center_axis',(0.,0.,-1.));
#138919=DIRECTION('ref_axis',(1.,1.03161403514696E-15,0.));
#138920=DIRECTION('',(1.,0.,0.));
#138921=DIRECTION('center_axis',(0.,0.,-1.));
#138922=DIRECTION('ref_axis',(1.,1.34109824569105E-14,0.));
#138923=DIRECTION('',(-0.819152044288992,0.573576436351045,0.));
#138924=DIRECTION('center_axis',(0.,0.,1.));
#138925=DIRECTION('ref_axis',(1.,0.,0.));
#138926=DIRECTION('center_axis',(0.,0.,-1.));
#138927=DIRECTION('ref_axis',(1.,0.,0.));
#138928=DIRECTION('center_axis',(0.,0.,1.));
#138929=DIRECTION('ref_axis',(1.,0.,0.));
#138930=DIRECTION('',(-0.819152044288992,-0.573576436351046,0.));
#138931=DIRECTION('center_axis',(-0.573576436351045,-0.819152044288992,
0.));
#138932=DIRECTION('ref_axis',(0.819152044288992,-0.573576436351045,0.));
#138933=DIRECTION('',(-0.819152044288992,0.573576436351045,0.));
#138934=DIRECTION('',(0.,0.,-1.));
#138935=DIRECTION('',(0.819152044288992,-0.573576436351045,0.));
#138936=DIRECTION('center_axis',(0.819152044288992,0.573576436351046,0.));
#138937=DIRECTION('ref_axis',(-0.573576436351046,0.819152044288992,0.));
#138938=DIRECTION('',(0.,0.,1.));
#138939=DIRECTION('',(0.573576436351046,-0.819152044288992,0.));
#138940=DIRECTION('',(-0.573576436351046,0.819152044288992,0.));
#138941=DIRECTION('center_axis',(0.,0.,1.));
#138942=DIRECTION('ref_axis',(1.,0.,0.));
#138943=DIRECTION('center_axis',(0.,0.,-1.));
#138944=DIRECTION('ref_axis',(1.,3.45590701774231E-14,0.));
#138945=DIRECTION('',(0.,1.,0.));
#138946=DIRECTION('center_axis',(0.,0.,-1.));
#138947=DIRECTION('ref_axis',(1.,0.,0.));
#138948=DIRECTION('',(-0.573576436351045,-0.819152044288992,0.));
#138949=DIRECTION('',(0.573576436351046,-0.819152044288992,0.));
#138950=DIRECTION('center_axis',(0.819152044288993,-0.573576436351045,0.));
#138951=DIRECTION('ref_axis',(0.573576436351045,0.819152044288992,0.));
#138952=DIRECTION('',(-0.573576436351045,-0.819152044288993,0.));
#138953=DIRECTION('center_axis',(0.819152044299452,-0.573576436336108,-7.19288685875037E-12));
#138954=DIRECTION('ref_axis',(0.573575979835469,0.819151392348989,-0.00126165307995225));
#138955=DIRECTION('',(0.,0.,-1.));
#138956=DIRECTION('',(0.573576436351045,0.819152044288992,0.));
#138957=DIRECTION('center_axis',(0.,0.,-1.));
#138958=DIRECTION('ref_axis',(-1.,0.,0.));
#138959=DIRECTION('center_axis',(0.,0.,1.));
#138960=DIRECTION('ref_axis',(1.,0.,0.));
#138961=DIRECTION('center_axis',(0.,0.,-1.));
#138962=DIRECTION('ref_axis',(-1.,0.,0.));
#138963=DIRECTION('center_axis',(0.,0.,-1.));
#138964=DIRECTION('ref_axis',(-1.,0.,0.));
#138965=DIRECTION('center_axis',(0.999699861223894,0.0244987210755295,1.16013489275163E-5));
#138966=DIRECTION('ref_axis',(-0.0243127779752216,0.992053772369109,0.123443110603017));
#138967=DIRECTION('center_axis',(0.,0.,-1.));
#138968=DIRECTION('ref_axis',(-1.,0.,0.));
#138969=DIRECTION('center_axis',(-0.999699861223916,0.0244987210746371,
1.16013488461091E-5));
#138970=DIRECTION('ref_axis',(0.0244987211028544,0.999699861287902,2.29639131106108E-6));
#138971=DIRECTION('center_axis',(0.,0.,-1.));
#138972=DIRECTION('ref_axis',(-1.,0.,0.));
#138973=DIRECTION('center_axis',(0.,0.,-1.));
#138974=DIRECTION('ref_axis',(1.,1.22464679914735E-16,0.));
#138975=DIRECTION('center_axis',(0.,0.,1.));
#138976=DIRECTION('ref_axis',(1.,0.,0.));
#138977=DIRECTION('center_axis',(0.,0.,-1.));
#138978=DIRECTION('ref_axis',(-1.,0.,0.));
#138979=DIRECTION('center_axis',(0.,0.,-1.));
#138980=DIRECTION('ref_axis',(1.,5.46369598732852E-15,0.));
#138981=DIRECTION('center_axis',(0.,0.,1.));
#138982=DIRECTION('ref_axis',(1.,0.,0.));
#138983=DIRECTION('center_axis',(0.,0.,-1.));
#138984=DIRECTION('ref_axis',(-1.,0.,0.));
#138985=DIRECTION('center_axis',(0.,0.,-1.));
#138986=DIRECTION('ref_axis',(1.,0.,0.));
#138987=DIRECTION('center_axis',(0.,0.,1.));
#138988=DIRECTION('ref_axis',(-0.986793248448819,-0.161984828968107,0.));
#138989=DIRECTION('center_axis',(0.,0.,-1.));
#138990=DIRECTION('ref_axis',(-1.,0.,0.));
#138991=DIRECTION('center_axis',(0.,0.,1.));
#138992=DIRECTION('ref_axis',(-0.986792877850041,0.161987086597769,0.));
#138993=DIRECTION('center_axis',(0.,0.,-1.));
#138994=DIRECTION('ref_axis',(-1.,0.,0.));
#138995=DIRECTION('center_axis',(0.,0.,1.));
#138996=DIRECTION('ref_axis',(1.,0.,0.));
#138997=DIRECTION('center_axis',(0.,0.,-1.));
#138998=DIRECTION('ref_axis',(-1.,0.,0.));
#138999=DIRECTION('center_axis',(0.,0.,1.));
#139000=DIRECTION('ref_axis',(1.,0.,0.));
#139001=DIRECTION('center_axis',(0.,0.,-1.));
#139002=DIRECTION('ref_axis',(-1.,0.,0.));
#139003=DIRECTION('center_axis',(0.950906387788118,0.309478661079813,0.));
#139004=DIRECTION('ref_axis',(-0.309478661079813,0.950906387788118,0.));
#139005=DIRECTION('center_axis',(-0.819152044288992,0.573576436351046,0.));
#139006=DIRECTION('ref_axis',(-0.573576436351046,-0.819152044288992,0.));
#139007=DIRECTION('center_axis',(-0.819152044288992,0.573576436351045,0.));
#139008=DIRECTION('ref_axis',(-0.573576436351045,-0.819152044288992,0.));
#139009=DIRECTION('center_axis',(-0.819152044288993,0.573576436351045,0.));
#139010=DIRECTION('ref_axis',(-0.573576436351045,-0.819152044288993,0.));
#139011=DIRECTION('center_axis',(0.,0.,1.));
#139012=DIRECTION('ref_axis',(1.,0.,0.));
#139013=DIRECTION('center_axis',(0.950906387788118,-0.309478661079813,0.));
#139014=DIRECTION('ref_axis',(0.309478661079813,0.950906387788118,0.));
#139015=DIRECTION('center_axis',(0.,0.,1.));
#139016=DIRECTION('ref_axis',(1.,0.,0.));
#139017=DIRECTION('center_axis',(-0.858390633711205,0.51299660813389,-6.25331394795773E-15));
#139018=DIRECTION('ref_axis',(-0.51299660813389,-0.858390633711205,-1.03337427582459E-31));
#139019=DIRECTION('center_axis',(0.819152044288993,0.573576436351045,0.));
#139020=DIRECTION('ref_axis',(-0.573576436351045,0.819152044288993,0.));
#139021=DIRECTION('center_axis',(-0.819152044288992,-0.573576436351046,
0.));
#139022=DIRECTION('ref_axis',(0.573576436351046,-0.819152044288992,0.));
#139023=DIRECTION('center_axis',(0.819152044288993,0.573576436351045,0.));
#139024=DIRECTION('ref_axis',(-0.573576436351045,0.819152044288993,0.));
#139025=DIRECTION('center_axis',(-1.,0.,0.));
#139026=DIRECTION('ref_axis',(0.,0.,1.));
#139027=DIRECTION('center_axis',(0.,0.,1.));
#139028=DIRECTION('ref_axis',(1.,0.,0.));
#139029=DIRECTION('center_axis',(0.858390633711208,0.512996608133885,0.));
#139030=DIRECTION('ref_axis',(-0.512996608133885,0.858390633711208,0.));
#139031=DIRECTION('center_axis',(-0.573576436351045,-0.819152044288993,
0.));
#139032=DIRECTION('ref_axis',(0.819152044288992,-0.573576436351045,0.));
#139033=DIRECTION('center_axis',(-0.573576436351045,-0.819152044288993,
0.));
#139034=DIRECTION('ref_axis',(0.819152044288993,-0.573576436351045,0.));
#139035=DIRECTION('center_axis',(0.,0.,1.));
#139036=DIRECTION('ref_axis',(1.,0.,0.));
#139037=DIRECTION('center_axis',(-0.51299660813389,-0.858390633711205,0.));
#139038=DIRECTION('ref_axis',(0.858390633711205,-0.51299660813389,0.));
#139039=DIRECTION('center_axis',(0.573576436351046,-0.819152044288992,0.));
#139040=DIRECTION('ref_axis',(0.819152044288992,0.573576436351046,0.));
#139041=DIRECTION('center_axis',(-0.573576436351045,0.819152044288993,0.));
#139042=DIRECTION('ref_axis',(-0.819152044288993,-0.573576436351045,0.));
#139043=DIRECTION('center_axis',(0.,-1.,0.));
#139044=DIRECTION('ref_axis',(0.,0.,-1.));
#139045=DIRECTION('center_axis',(0.,0.,1.));
#139046=DIRECTION('ref_axis',(1.,0.,0.));
#139047=DIRECTION('center_axis',(-0.51299660813389,0.858390633711205,0.));
#139048=DIRECTION('ref_axis',(-0.858390633711205,-0.51299660813389,0.));
#139049=DIRECTION('center_axis',(0.573576436351045,0.819152044288992,0.));
#139050=DIRECTION('ref_axis',(-0.819152044288992,0.573576436351045,0.));
#139051=DIRECTION('center_axis',(0.573576436351045,0.819152044288993,0.));
#139052=DIRECTION('ref_axis',(-0.819152044288993,0.573576436351045,0.));
#139053=DIRECTION('center_axis',(0.,0.,1.));
#139054=DIRECTION('ref_axis',(-1.,-1.22464679914735E-16,0.));
#139055=DIRECTION('center_axis',(0.,0.,1.));
#139056=DIRECTION('ref_axis',(1.,0.,0.));
#139057=DIRECTION('center_axis',(0.51299660813389,0.858390633711205,0.));
#139058=DIRECTION('ref_axis',(-0.858390633711205,0.51299660813389,0.));
#139059=DIRECTION('center_axis',(-0.573576436351045,0.819152044288992,0.));
#139060=DIRECTION('ref_axis',(-0.819152044288992,-0.573576436351045,0.));
#139061=DIRECTION('center_axis',(0.573576436351045,-0.819152044288993,0.));
#139062=DIRECTION('ref_axis',(0.819152044288993,0.573576436351045,0.));
#139063=DIRECTION('center_axis',(0.,1.,0.));
#139064=DIRECTION('ref_axis',(0.,0.,1.));
#139065=DIRECTION('center_axis',(0.,0.,1.));
#139066=DIRECTION('ref_axis',(1.,0.,0.));
#139067=DIRECTION('center_axis',(0.51299660813389,-0.858390633711205,0.));
#139068=DIRECTION('ref_axis',(0.858390633711205,0.51299660813389,0.));
#139069=DIRECTION('center_axis',(1.,0.,0.));
#139070=DIRECTION('ref_axis',(0.,0.,-1.));
#139071=DIRECTION('center_axis',(-1.,0.,0.));
#139072=DIRECTION('ref_axis',(0.,0.,-1.));
#139073=DIRECTION('center_axis',(-0.926843172992801,0.,-0.37544870844982));
#139074=DIRECTION('ref_axis',(-0.37544870844982,0.,0.926843172992801));
#139075=DIRECTION('center_axis',(0.926843172992801,0.,-0.37544870844982));
#139076=DIRECTION('ref_axis',(0.37544870844982,0.,0.926843172992801));
#139077=DIRECTION('center_axis',(1.,0.,0.));
#139078=DIRECTION('ref_axis',(0.,0.,-1.));
#139079=DIRECTION('center_axis',(1.,0.,0.));
#139080=DIRECTION('ref_axis',(0.,0.,-1.));
#139081=DIRECTION('center_axis',(0.573576436351045,-0.819152044288992,0.));
#139082=DIRECTION('ref_axis',(-0.57922836252423,-0.405580065784332,0.707106296313275));
#139083=DIRECTION('center_axis',(-0.573576436351042,0.819152044288994,0.));
#139084=DIRECTION('ref_axis',(-0.819152044288994,-0.573576436351042,0.));
#139085=DIRECTION('center_axis',(0.,0.,1.));
#139086=DIRECTION('ref_axis',(-0.707106781186548,0.707106781186548,0.));
#139087=DIRECTION('center_axis',(0.819152044288994,-0.573576436351042,0.));
#139088=DIRECTION('ref_axis',(0.573576436351042,0.819152044288994,0.));
#139089=DIRECTION('center_axis',(-0.819152044288992,0.573576436351046,0.));
#139090=DIRECTION('ref_axis',(0.405580057474329,0.579228350656315,0.707106310801343));
#139091=DIRECTION('center_axis',(-0.819152044288992,-0.573576436351046,
0.));
#139092=DIRECTION('ref_axis',(-0.40558006578429,0.579228362524169,0.707106296313348));
#139093=DIRECTION('center_axis',(0.573576436351045,0.819152044288993,0.));
#139094=DIRECTION('ref_axis',(0.579228271576628,-0.405580002102135,0.707106407339931));
#139095=DIRECTION('center_axis',(-0.573576436351046,0.819152044288992,0.));
#139096=DIRECTION('ref_axis',(0.579228362524086,0.405580065784232,0.70710629631345));
#139097=DIRECTION('center_axis',(0.819152044288992,-0.573576436351045,0.));
#139098=DIRECTION('ref_axis',(-0.405580057474373,-0.579228350656379,0.707106310801265));
#139099=DIRECTION('center_axis',(0.819152044288992,0.573576436351046,0.));
#139100=DIRECTION('ref_axis',(0.405580065784262,-0.579228362524129,0.707106296313398));
#139101=DIRECTION('center_axis',(-0.819152044288994,-0.573576436351042,
0.));
#139102=DIRECTION('ref_axis',(0.573576436351042,-0.819152044288994,0.));
#139103=DIRECTION('center_axis',(0.,0.,1.));
#139104=DIRECTION('ref_axis',(-0.707106781186547,-0.707106781186548,0.));
#139105=DIRECTION('center_axis',(0.573576436351042,0.819152044288994,0.));
#139106=DIRECTION('ref_axis',(-0.819152044288994,0.573576436351042,0.));
#139107=DIRECTION('center_axis',(-0.573576436351045,-0.819152044288992,
0.));
#139108=DIRECTION('ref_axis',(-0.579228350656326,0.405580057474336,0.70710631080133));
#139109=DIRECTION('center_axis',(0.932736302061011,-0.360559275040251,3.939972528463E-15));
#139110=DIRECTION('ref_axis',(0.360559275040251,0.932736302061011,-2.72809344998311E-30));
#139111=DIRECTION('center_axis',(0.,0.,1.));
#139112=DIRECTION('ref_axis',(1.,0.,0.));
#139113=DIRECTION('center_axis',(0.360559275040245,-0.932736302061013,0.));
#139114=DIRECTION('ref_axis',(0.932736302061013,0.360559275040245,0.));
#139115=DIRECTION('center_axis',(0.36055927504025,0.932736302061011,-1.9699862642315E-15));
#139116=DIRECTION('ref_axis',(-0.932736302061011,0.36055927504025,4.58218097742534E-31));
#139117=DIRECTION('center_axis',(0.,0.,1.));
#139118=DIRECTION('ref_axis',(1.,0.,0.));
#139119=DIRECTION('center_axis',(0.932736302061012,0.360559275040248,0.));
#139120=DIRECTION('ref_axis',(-0.360559275040248,0.932736302061012,0.));
#139121=DIRECTION('center_axis',(-0.932736302061006,0.360559275040262,9.03616011926949E-15));
#139122=DIRECTION('ref_axis',(-0.360559275040262,-0.932736302061006,-4.62325821272544E-30));
#139123=DIRECTION('center_axis',(0.,0.,1.));
#139124=DIRECTION('ref_axis',(1.,0.,0.));
#139125=DIRECTION('center_axis',(-0.360559275040266,0.932736302061005,0.));
#139126=DIRECTION('ref_axis',(-0.932736302061005,-0.360559275040266,0.));
#139127=DIRECTION('center_axis',(-0.524947284506131,0.698415662498183,-0.486462651050277));
#139128=DIRECTION('ref_axis',(0.477697561100747,0.714799658786074,0.510750905939197));
#139129=DIRECTION('center_axis',(0.932736302061011,0.36055927504025,0.));
#139130=DIRECTION('ref_axis',(-0.36055927504025,0.932736302061011,0.));
#139131=DIRECTION('center_axis',(0.,0.,1.));
#139132=DIRECTION('ref_axis',(1.,0.,0.));
#139133=DIRECTION('center_axis',(0.36055927504025,0.932736302061011,-6.37023448850799E-15));
#139134=DIRECTION('ref_axis',(-0.932736302061011,0.36055927504025,-9.63555131444101E-31));
#139135=DIRECTION('center_axis',(0.,-0.1229930844099,0.992407527776437));
#139136=DIRECTION('ref_axis',(0.,-0.992407527776437,-0.1229930844099));
#139137=DIRECTION('center_axis',(0.,0.,1.));
#139138=DIRECTION('ref_axis',(1.,0.,0.));
#139139=DIRECTION('center_axis',(0.,0.,1.));
#139140=DIRECTION('ref_axis',(-0.753587189137082,-0.65734796597272,0.));
#139141=DIRECTION('center_axis',(0.,-0.122993084409903,0.992407527776437));
#139142=DIRECTION('ref_axis',(0.,-0.992407527776436,-0.122993084409903));
#139143=DIRECTION('center_axis',(0.,0.,1.));
#139144=DIRECTION('ref_axis',(1.,0.,0.));
#139145=DIRECTION('center_axis',(0.,0.,1.));
#139146=DIRECTION('ref_axis',(1.,0.,0.));
#139147=DIRECTION('center_axis',(0.29613474068235,0.955146174865919,-1.60736624536386E-14));
#139148=DIRECTION('ref_axis',(-0.955146174865919,0.29613474068235,-1.70032019875616E-29));
#139149=DIRECTION('center_axis',(0.,1.,0.));
#139150=DIRECTION('ref_axis',(1.,0.,0.));
#139151=DIRECTION('center_axis',(-0.296134740682398,0.955146174865905,0.));
#139152=DIRECTION('ref_axis',(-0.955146174865904,-0.296134740682398,0.));
#139153=DIRECTION('center_axis',(0.,1.,0.));
#139154=DIRECTION('ref_axis',(1.,0.,0.));
#139155=DIRECTION('center_axis',(0.14289314960746,0.192051979157228,0.970926148116865));
#139156=DIRECTION('ref_axis',(-1.42059255304153E-13,0.980992979553962,-0.194043227312473));
#139157=DIRECTION('center_axis',(0.134462341405205,-0.839995008085521,0.525669349625063));
#139158=DIRECTION('ref_axis',(-1.06456783153248E-16,-0.530486857586963,
-0.847693160245799));
#139159=DIRECTION('center_axis',(0.120848057364438,-0.6566208576434,0.744476189235685));
#139160=DIRECTION('ref_axis',(-7.75623579529732E-17,-0.749972726964935,
-0.661468751195987));
#139161=DIRECTION('center_axis',(-0.839995008085506,0.13446234140521,0.525669349625084));
#139162=DIRECTION('ref_axis',(0.530486857586985,7.38424576160362E-17,0.847693160245785));
#139163=DIRECTION('center_axis',(-0.656620857643591,0.120848057364596,0.744476189235491));
#139164=DIRECTION('ref_axis',(0.749972726964755,5.96486641503031E-17,0.661468751196192));
#139165=DIRECTION('center_axis',(0.839995008085611,0.134462341405169,0.525669349624927));
#139166=DIRECTION('ref_axis',(0.530486857586823,-1.49812135928454E-16,-0.847693160245886));
#139167=DIRECTION('center_axis',(0.65662085764469,0.120848057364753,0.744476189234497));
#139168=DIRECTION('ref_axis',(0.749972726963767,6.2356189333396E-17,-0.661468751197311));
#139169=DIRECTION('center_axis',(-0.134462341405213,-0.839995008085543,
0.525669349625026));
#139170=DIRECTION('ref_axis',(-1.21569156643707E-16,-0.530486857586926,
-0.847693160245822));
#139171=DIRECTION('center_axis',(-0.120848057364571,-0.656620857643531,
0.744476189235548));
#139172=DIRECTION('ref_axis',(3.55024582468309E-17,-0.74997272696481,-0.661468751196129));
#139173=DIRECTION('center_axis',(-0.134462341405157,0.839995008085507,0.525669349625097));
#139174=DIRECTION('ref_axis',(6.43633176795525E-17,-0.530486857586994,0.847693160245779));
#139175=DIRECTION('center_axis',(-0.120848057364642,0.656620857644208,0.744476189234939));
#139176=DIRECTION('ref_axis',(-5.23473322259609E-17,-0.749972726964203,
0.661468751196817));
#139177=DIRECTION('center_axis',(0.839995008085624,-0.134462341405244,0.525669349624888));
#139178=DIRECTION('ref_axis',(0.530486857586789,-2.55916400237815E-17,-0.847693160245908));
#139179=DIRECTION('center_axis',(0.656620857643605,-0.120848057364609,0.744476189235477));
#139180=DIRECTION('ref_axis',(0.749972726964742,-6.28921792063169E-17,-0.661468751196207));
#139181=DIRECTION('center_axis',(0.65662085764265,0.120848057364237,-0.744476189236379));
#139182=DIRECTION('ref_axis',(-0.749972726965616,-9.44663393319256E-17,
-0.661468751195215));
#139183=DIRECTION('center_axis',(0.839995008085555,0.134462341405231,-0.525669349625));
#139184=DIRECTION('ref_axis',(-0.530486857586902,2.38349706059343E-16,-0.847693160245837));
#139185=DIRECTION('center_axis',(0.134462341405206,0.839995008085575,0.525669349624976));
#139186=DIRECTION('ref_axis',(1.44832680552187E-16,-0.530486857586875,0.847693160245854));
#139187=DIRECTION('center_axis',(0.12084805736459,0.656620857643582,0.7444761892355));
#139188=DIRECTION('ref_axis',(-8.18770910965257E-17,-0.749972726964763,
0.661468751196182));
#139189=DIRECTION('center_axis',(1.09273919746571E-14,1.,0.));
#139190=DIRECTION('ref_axis',(-1.,1.09273919746571E-14,0.));
#139191=DIRECTION('center_axis',(0.,-1.,0.));
#139192=DIRECTION('ref_axis',(0.,0.,-1.));
#139193=DIRECTION('center_axis',(0.,1.,0.));
#139194=DIRECTION('ref_axis',(0.,0.,1.));
#139195=DIRECTION('center_axis',(0.,0.,1.));
#139196=DIRECTION('ref_axis',(1.,0.,0.));
#139197=DIRECTION('center_axis',(0.,1.,0.));
#139198=DIRECTION('ref_axis',(0.,0.,1.));
#139199=DIRECTION('center_axis',(-1.,0.,0.));
#139200=DIRECTION('ref_axis',(0.,1.,0.));
#139201=DIRECTION('center_axis',(0.,0.,1.));
#139202=DIRECTION('ref_axis',(0.,-1.,0.));
#139203=DIRECTION('center_axis',(0.0871557427476584,-0.996194698091746,
0.));
#139204=DIRECTION('ref_axis',(0.996194698091746,0.0871557427476567,0.));
#139205=DIRECTION('center_axis',(0.0871557427476584,-0.996194698091746,
0.));
#139206=DIRECTION('ref_axis',(0.996194698091746,0.0871557427476584,0.));
#139207=DIRECTION('center_axis',(0.,0.,-1.));
#139208=DIRECTION('ref_axis',(-0.996194698091746,-0.0871557427476585,0.));
#139209=DIRECTION('center_axis',(-0.0871557427476584,0.996194698091746,
0.));
#139210=DIRECTION('ref_axis',(0.996194698091745,0.0871557427476584,0.));
#139211=DIRECTION('center_axis',(0.0871557427476584,-0.996194698091746,
0.));
#139212=DIRECTION('ref_axis',(0.996194698091746,0.0871557427476584,0.));
#139213=DIRECTION('center_axis',(-0.0871557427476584,0.996194698091746,
1.2273002111418E-17));
#139214=DIRECTION('ref_axis',(-0.996194698091746,-0.0871557427476567,0.));
#139215=DIRECTION('center_axis',(-0.0871557427476584,0.996194698091746,
1.2273002111418E-17));
#139216=DIRECTION('ref_axis',(-0.996194698091746,-0.0871557427476584,-1.17790383141732E-32));
#139217=DIRECTION('center_axis',(-1.06966261476422E-18,1.22262996330634E-17,
-1.));
#139218=DIRECTION('ref_axis',(0.996194698091746,0.0871557427476585,0.));
#139219=DIRECTION('center_axis',(0.0871557427476584,-0.996194698091746,
-1.2273002111418E-17));
#139220=DIRECTION('ref_axis',(-0.996194698091746,-0.0871557427476584,3.71474908964093E-32));
#139221=DIRECTION('center_axis',(-0.0871557427476584,0.996194698091746,
1.2273002111418E-17));
#139222=DIRECTION('ref_axis',(-0.996194698091746,-0.0871557427476584,-1.17790383141732E-32));
#139223=DIRECTION('center_axis',(-0.990322420104686,-0.0881064801885017,
0.107232235763274));
#139224=DIRECTION('ref_axis',(0.107650883357545,-1.2725694566787E-17,0.994188758391655));
#139225=DIRECTION('center_axis',(0.087146257713358,-0.996105346075413,0.0134040772356536));
#139226=DIRECTION('ref_axis',(-0.00117066129865813,0.0133528590446799,0.999910161318234));
#139227=DIRECTION('center_axis',(0.990557289919919,0.0851973867025048,-0.107413503273888));
#139228=DIRECTION('ref_axis',(-0.107805473979535,-3.10296312186364E-18,
-0.994172007139634));
#139229=DIRECTION('center_axis',(-4.73068525233381E-16,6.98056821064309E-15,
-1.));
#139230=DIRECTION('ref_axis',(-0.0871557427476583,0.996194698091746,6.99523567979768E-15));
#139231=DIRECTION('center_axis',(-0.0871557427476584,0.996194698091746,
1.2273002111418E-17));
#139232=DIRECTION('ref_axis',(1.06966261476422E-18,-1.22262996330634E-17,
1.));
#139233=DIRECTION('center_axis',(0.0871557427476584,-0.996194698091746,
-1.2273002111418E-17));
#139234=DIRECTION('ref_axis',(-1.06966261476422E-18,1.22262996330634E-17,
-1.));
#139235=DIRECTION('',(0.0871557427476584,-0.996194698091746,-1.2273002111418E-17));
#139236=DIRECTION('center_axis',(-0.0869877574560655,0.996034814013987,
0.0186488424543453));
#139237=DIRECTION('ref_axis',(-0.109438987085954,0.00905210098230124,-0.993952296427453));
#139238=DIRECTION('center_axis',(0.0871557427476584,-0.996194698091746,
-1.2273002111418E-17));
#139239=DIRECTION('ref_axis',(-1.06966261476421E-18,1.22262996330634E-17,
-1.));
#139240=DIRECTION('',(-0.0871557427476584,0.996194698091746,1.2273002111418E-17));
#139241=DIRECTION('center_axis',(-0.0871557427476583,0.996194698091746,
0.));
#139242=DIRECTION('ref_axis',(0.996194698091745,0.08715574274766,0.));
#139243=DIRECTION('center_axis',(1.75242621800742E-16,3.01185978847313E-18,
1.));
#139244=DIRECTION('ref_axis',(-0.996194698091746,-0.0871557427476572,1.74838271594512E-16));
#139245=DIRECTION('center_axis',(-0.0871557427476584,0.996194698091746,
1.2273002111418E-17));
#139246=DIRECTION('ref_axis',(5.35850844502666E-19,-1.2273002111418E-17,
1.));
#139247=DIRECTION('center_axis',(-4.73068525233381E-16,6.98056821064309E-15,
-1.));
#139248=DIRECTION('ref_axis',(0.,1.,6.98056225145764E-15));
#139249=DIRECTION('center_axis',(-4.73068525233381E-16,6.98056821064309E-15,
-1.));
#139250=DIRECTION('ref_axis',(-1.72250008496352E-34,1.,6.98056821064309E-15));
#139251=DIRECTION('center_axis',(-1.,1.22464679914732E-16,4.73068525233382E-16));
#139252=DIRECTION('ref_axis',(-1.22464679914735E-16,-1.,-6.98139884808413E-15));
#139253=DIRECTION('center_axis',(4.73068525233381E-16,-6.98056821064309E-15,
1.));
#139254=DIRECTION('ref_axis',(-3.49817812003891E-35,1.,6.98056821064309E-15));
#139255=DIRECTION('center_axis',(-4.73068525233381E-16,6.98056821064309E-15,
-1.));
#139256=DIRECTION('ref_axis',(-1.72250008496352E-34,1.,6.98056821064309E-15));
#139257=DIRECTION('center_axis',(-4.73068525233381E-16,6.98056821064309E-15,
-1.));
#139258=DIRECTION('ref_axis',(0.,1.,6.98058702583013E-15));
#139259=DIRECTION('center_axis',(-4.73068525233381E-16,6.98056821064309E-15,
-1.));
#139260=DIRECTION('ref_axis',(1.01760986150651E-34,1.,6.98056821064309E-15));
#139261=DIRECTION('center_axis',(-1.,1.22464679914732E-16,4.73068525233382E-16));
#139262=DIRECTION('ref_axis',(-1.22464679914735E-16,-1.,-6.98058702583013E-15));
#139263=DIRECTION('center_axis',(4.73068525233381E-16,-6.98056821064309E-15,
1.));
#139264=DIRECTION('ref_axis',(2.37981304966787E-34,1.,6.98056821064309E-15));
#139265=DIRECTION('center_axis',(4.73068525233381E-16,-6.98056821064309E-15,
1.));
#139266=DIRECTION('ref_axis',(2.37981304966787E-34,1.,6.98056821064309E-15));
#139267=DIRECTION('center_axis',(-0.0871557427476584,0.996194698091746,
1.2273002111418E-17));
#139268=DIRECTION('ref_axis',(1.06966261476422E-18,-1.22262996330634E-17,
1.));
#139269=DIRECTION('',(-0.0871557427476584,0.996194698091746,1.2273002111418E-17));
#139270=DIRECTION('center_axis',(-4.73068525233381E-16,6.98056821064309E-15,
-1.));
#139271=DIRECTION('ref_axis',(-0.0871557427476584,0.996194698091745,6.99523567979768E-15));
#139272=DIRECTION('center_axis',(-4.73068525233381E-16,6.98056821064309E-15,
-1.));
#139273=DIRECTION('ref_axis',(-0.0871557427476584,0.996194698091745,6.99523567979768E-15));
#139274=DIRECTION('',(-4.73068525233381E-16,6.98056821064309E-15,-1.));
#139275=DIRECTION('center_axis',(-4.73068525233381E-16,6.98056821064309E-15,
-1.));
#139276=DIRECTION('ref_axis',(-0.0871557427476584,0.996194698091745,6.99523567979768E-15));
#139277=DIRECTION('',(4.73068525233381E-16,-6.98056821064309E-15,1.));
#139278=DIRECTION('center_axis',(-4.73068525233381E-16,6.98056821064309E-15,
-1.));
#139279=DIRECTION('ref_axis',(-0.996194698091745,-0.0871557427476584,-1.37128250527716E-16));
#139280=DIRECTION('center_axis',(-4.73068525233381E-16,6.98056821064309E-15,
-1.));
#139281=DIRECTION('ref_axis',(-0.0871557427476584,0.996194698091746,6.99523567979768E-15));
#139282=DIRECTION('center_axis',(-4.73068525233381E-16,6.98056821064309E-15,
-1.));
#139283=DIRECTION('ref_axis',(-0.0871557427476584,0.996194698091746,6.99523567979768E-15));
#139284=DIRECTION('center_axis',(1.4081690688991E-16,0.,1.));
#139285=DIRECTION('ref_axis',(1.,0.,-1.25828382064365E-16));
#139286=DIRECTION('center_axis',(1.4081690688991E-16,0.,1.));
#139287=DIRECTION('ref_axis',(1.,0.,-1.4081690688991E-16));
#139288=DIRECTION('center_axis',(-1.22464679914735E-16,1.,1.7245097428856E-32));
#139289=DIRECTION('ref_axis',(-1.,-1.22464679914735E-16,1.57285477580457E-16));
#139290=DIRECTION('center_axis',(-1.4081690688991E-16,0.,-1.));
#139291=DIRECTION('ref_axis',(1.,0.,-1.4081690688991E-16));
#139292=DIRECTION('center_axis',(0.,0.,1.));
#139293=DIRECTION('ref_axis',(1.,0.,0.));
#139294=DIRECTION('center_axis',(0.,0.,1.));
#139295=DIRECTION('ref_axis',(1.,0.,0.));
#139296=DIRECTION('center_axis',(1.22464679914735E-16,-1.,0.));
#139297=DIRECTION('ref_axis',(-1.,-1.22464679914735E-16,0.));
#139298=DIRECTION('center_axis',(0.,0.,-1.));
#139299=DIRECTION('ref_axis',(1.,0.,0.));
#139300=DIRECTION('center_axis',(0.,0.,-1.));
#139301=DIRECTION('ref_axis',(1.,0.,0.));
#139302=DIRECTION('center_axis',(0.,0.,1.));
#139303=DIRECTION('ref_axis',(1.,0.,0.));
#139304=DIRECTION('center_axis',(0.,0.,1.));
#139305=DIRECTION('ref_axis',(1.,0.,0.));
#139306=DIRECTION('center_axis',(0.,0.,1.));
#139307=DIRECTION('ref_axis',(1.,0.,0.));
#139308=DIRECTION('center_axis',(1.22464679914735E-16,-1.,0.));
#139309=DIRECTION('ref_axis',(-1.,-1.22464679914735E-16,0.));
#139310=DIRECTION('center_axis',(0.,0.,-1.));
#139311=DIRECTION('ref_axis',(1.,0.,0.));
#139312=DIRECTION('center_axis',(1.4081690688991E-16,0.,1.));
#139313=DIRECTION('ref_axis',(1.,0.,-1.24674611521858E-16));
#139314=DIRECTION('center_axis',(1.4081690688991E-16,0.,1.));
#139315=DIRECTION('ref_axis',(-1.,0.,1.4081690688991E-16));
#139316=DIRECTION('center_axis',(1.22464679914735E-16,-1.,-1.7245097428856E-32));
#139317=DIRECTION('ref_axis',(-1.,-1.22464679914735E-16,1.55843264402323E-16));
#139318=DIRECTION('center_axis',(-1.4081690688991E-16,0.,-1.));
#139319=DIRECTION('ref_axis',(1.,0.,-1.4081690688991E-16));
#139320=DIRECTION('center_axis',(1.4081690688991E-16,0.,1.));
#139321=DIRECTION('ref_axis',(1.,0.,-1.23223868360489E-16));
#139322=DIRECTION('center_axis',(1.4081690688991E-16,0.,1.));
#139323=DIRECTION('ref_axis',(1.,0.,-1.4081690688991E-16));
#139324=DIRECTION('center_axis',(1.22464679914735E-16,-1.,-1.7245097428856E-32));
#139325=DIRECTION('ref_axis',(-1.,-1.22464679914735E-16,1.54029835450611E-16));
#139326=DIRECTION('center_axis',(-1.4081690688991E-16,0.,-1.));
#139327=DIRECTION('ref_axis',(-1.,0.,1.4081690688991E-16));
#139328=DIRECTION('center_axis',(1.4081690688991E-16,0.,1.));
#139329=DIRECTION('ref_axis',(1.,0.,-1.4081690688991E-16));
#139330=DIRECTION('center_axis',(1.4081690688991E-16,0.,1.));
#139331=DIRECTION('ref_axis',(1.,0.,-1.4081690688991E-16));
#139332=DIRECTION('',(-1.40816906889911E-16,0.,-1.));
#139333=DIRECTION('center_axis',(1.4081690688991E-16,0.,1.));
#139334=DIRECTION('ref_axis',(1.,0.,-1.4081690688991E-16));
#139335=DIRECTION('center_axis',(1.4081690688991E-16,0.,1.));
#139336=DIRECTION('ref_axis',(1.,0.,-1.4081690688991E-16));
#139337=DIRECTION('',(-0.5299192642332,-6.48963930749709E-17,0.848048096156429));
#139338=DIRECTION('center_axis',(1.4081690688991E-16,0.,1.));
#139339=DIRECTION('ref_axis',(1.,0.,-1.4081690688991E-16));
#139340=DIRECTION('',(0.529919264233204,6.48963930749714E-17,-0.848048096156427));
#139341=DIRECTION('center_axis',(0.,0.,-1.));
#139342=DIRECTION('ref_axis',(-1.,0.,0.));
#139343=DIRECTION('center_axis',(1.4081690688991E-16,0.,1.));
#139344=DIRECTION('ref_axis',(1.,0.,-1.4081690688991E-16));
#139345=DIRECTION('',(0.,0.,1.));
#139346=DIRECTION('center_axis',(0.,0.,-1.));
#139347=DIRECTION('ref_axis',(-1.,0.,0.));
#139348=DIRECTION('',(0.,0.,-1.));
#139349=DIRECTION('center_axis',(0.,0.,-1.));
#139350=DIRECTION('ref_axis',(-1.,0.,0.));
#139351=DIRECTION('center_axis',(0.,0.,-1.));
#139352=DIRECTION('ref_axis',(-1.,0.,0.));
#139353=DIRECTION('center_axis',(0.,0.,-1.));
#139354=DIRECTION('ref_axis',(-1.,0.,0.));
#139355=DIRECTION('',(0.,0.,1.));
#139356=DIRECTION('center_axis',(0.,0.,-1.));
#139357=DIRECTION('ref_axis',(1.,0.,0.));
#139358=DIRECTION('center_axis',(0.,0.,1.));
#139359=DIRECTION('ref_axis',(1.,0.,0.));
#139360=DIRECTION('center_axis',(0.,0.,-1.));
#139361=DIRECTION('ref_axis',(-1.,0.,0.));
#139362=DIRECTION('center_axis',(0.,0.,1.));
#139363=DIRECTION('ref_axis',(1.,0.,0.));
#139364=DIRECTION('center_axis',(1.4081690688991E-16,0.,1.));
#139365=DIRECTION('ref_axis',(1.,0.,-1.40816906889911E-16));
#139366=DIRECTION('center_axis',(1.4081690688991E-16,0.,1.));
#139367=DIRECTION('ref_axis',(1.,0.,-1.40816906889911E-16));
#139368=DIRECTION('center_axis',(1.,-1.90843891001168E-31,-2.61618113230267E-16));
#139369=DIRECTION('ref_axis',(0.,1.,0.));
#139370=DIRECTION('',(1.,-1.90843891001168E-31,-2.61618113230267E-16));
#139371=DIRECTION('center_axis',(-1.,3.57620498399058E-12,-7.43666695244082E-12));
#139372=DIRECTION('ref_axis',(8.25152405459824E-12,0.441542383644494,-0.897240393342575));
#139373=DIRECTION('center_axis',(1.,-1.90843891001168E-31,-2.61618113230267E-16));
#139374=DIRECTION('ref_axis',(0.,1.,0.));
#139375=DIRECTION('',(1.,-1.90843891001168E-31,-2.61618113230267E-16));
#139376=DIRECTION('center_axis',(1.,-1.90843891001168E-31,-2.61618113230267E-16));
#139377=DIRECTION('ref_axis',(0.,1.,0.));
#139378=DIRECTION('',(1.,-1.90843891001168E-31,-2.61618113230267E-16));
#139379=DIRECTION('center_axis',(1.,-1.90843891001168E-31,-2.61618113230267E-16));
#139380=DIRECTION('ref_axis',(0.,1.,0.));
#139381=DIRECTION('',(1.,-1.90843891001168E-31,-2.61618113230267E-16));
#139382=DIRECTION('center_axis',(1.,-1.90843891001168E-31,-2.61618113230267E-16));
#139383=DIRECTION('ref_axis',(0.,1.,0.));
#139384=DIRECTION('',(1.,-1.90843891001168E-31,-2.61618113230267E-16));
#139385=DIRECTION('center_axis',(1.,-1.90843891001168E-31,-2.61618113230267E-16));
#139386=DIRECTION('ref_axis',(0.,1.,0.));
#139387=DIRECTION('',(1.,-1.90843891001168E-31,-2.61618113230267E-16));
#139388=DIRECTION('center_axis',(1.,-3.49148133884313E-15,0.));
#139389=DIRECTION('ref_axis',(0.,0.,1.));
#139390=DIRECTION('',(-1.,3.49148133884313E-15,0.));
#139391=DIRECTION('center_axis',(1.,-3.49148133884313E-15,0.));
#139392=DIRECTION('ref_axis',(0.,0.,1.));
#139393=DIRECTION('center_axis',(1.,-3.49148133884313E-15,0.));
#139394=DIRECTION('ref_axis',(0.,0.,1.));
#139395=DIRECTION('',(-1.,3.49148133884313E-15,0.));
#139396=DIRECTION('center_axis',(1.,-3.49148133884313E-15,0.));
#139397=DIRECTION('ref_axis',(0.,0.,1.));
#139398=DIRECTION('center_axis',(1.,-3.49148133884313E-15,0.));
#139399=DIRECTION('ref_axis',(0.,0.,1.));
#139400=DIRECTION('',(-1.,3.49148133884313E-15,0.));
#139401=DIRECTION('center_axis',(1.,-3.49148133884313E-15,0.));
#139402=DIRECTION('ref_axis',(0.,0.,1.));
#139403=DIRECTION('',(-1.,3.49148133884313E-15,0.));
#139404=DIRECTION('center_axis',(1.,-3.49148133884313E-15,0.));
#139405=DIRECTION('ref_axis',(0.,0.,1.));
#139406=DIRECTION('',(-1.,3.49148133884313E-15,0.));
#139407=DIRECTION('center_axis',(1.,-3.49148133884313E-15,0.));
#139408=DIRECTION('ref_axis',(0.,0.,1.));
#139409=DIRECTION('',(-1.,3.49148133884313E-15,0.));
#139410=DIRECTION('center_axis',(1.,-3.49148133884313E-15,0.));
#139411=DIRECTION('ref_axis',(0.,0.,1.));
#139412=DIRECTION('',(-1.,3.49148133884313E-15,0.));
#139413=DIRECTION('center_axis',(1.,-3.49148133884313E-15,0.));
#139414=DIRECTION('ref_axis',(0.,0.,1.));
#139415=DIRECTION('',(-1.,3.49148133884313E-15,0.));
#139416=DIRECTION('center_axis',(-1.,3.49148133884313E-15,0.));
#139417=DIRECTION('ref_axis',(0.,0.,1.));
#139418=DIRECTION('center_axis',(1.,-3.49148133884313E-15,0.));
#139419=DIRECTION('ref_axis',(0.,0.,1.));
#139420=DIRECTION('center_axis',(0.999733823610252,-0.00785201424948982,
0.0216939577268001));
#139421=DIRECTION('ref_axis',(0.000790766294128704,-0.928088776890918,-0.37235815674937));
#139422=DIRECTION('center_axis',(1.,7.68190179945482E-12,1.14262706414629E-12));
#139423=DIRECTION('ref_axis',(-4.47582277062776E-14,-0.141421341569384,
0.989949495756584));
#139424=DIRECTION('center_axis',(-0.99643212438083,0.0191622394024502,-0.0821938567229316));
#139425=DIRECTION('ref_axis',(-0.015721416758303,-0.998980952014553,-0.0423071455809782));
#139426=DIRECTION('',(-0.707106781186546,2.38225452545871E-15,0.707106781186549));
#139427=DIRECTION('center_axis',(-1.,3.49148133884313E-15,0.));
#139428=DIRECTION('ref_axis',(0.,0.,1.));
#139429=DIRECTION('center_axis',(-1.,3.49148133884313E-15,0.));
#139430=DIRECTION('ref_axis',(0.,0.,-1.));
#139431=DIRECTION('center_axis',(-1.,3.49148133884313E-15,0.));
#139432=DIRECTION('ref_axis',(0.,0.,1.));
#139433=DIRECTION('center_axis',(-0.999731535326071,-0.0209809681761542,
-0.00983139099868423));
#139434=DIRECTION('ref_axis',(-0.00512812960574839,-0.213430275538391,0.976944839676403));
#139435=DIRECTION('center_axis',(0.996321406376314,0.0724020542568729,0.0458431863607806));
#139436=DIRECTION('ref_axis',(-0.000636379506200249,-0.528690912836352,
0.848814180904978));
#139437=DIRECTION('center_axis',(-1.,3.49148133884313E-15,0.));
#139438=DIRECTION('ref_axis',(0.,0.,1.));
#139439=DIRECTION('',(0.707106781186545,-2.55544573670581E-15,-0.70710678118655));
#139440=DIRECTION('center_axis',(1.,-3.49148133884313E-15,0.));
#139441=DIRECTION('ref_axis',(0.,0.,1.));
#139442=DIRECTION('center_axis',(1.,-3.49148133884313E-15,0.));
#139443=DIRECTION('ref_axis',(0.,0.,1.));
#139444=DIRECTION('center_axis',(1.,-3.49148133884313E-15,0.));
#139445=DIRECTION('ref_axis',(0.,0.,1.));
#139446=DIRECTION('center_axis',(1.,-3.49148133884313E-15,0.));
#139447=DIRECTION('ref_axis',(0.,0.,1.));
#139448=DIRECTION('center_axis',(1.,-3.49148133884313E-15,0.));
#139449=DIRECTION('ref_axis',(0.,0.,1.));
#139450=DIRECTION('center_axis',(1.,-3.49148133884313E-15,0.));
#139451=DIRECTION('ref_axis',(0.,0.,1.));
#139452=DIRECTION('center_axis',(1.,-3.49148133884313E-15,0.));
#139453=DIRECTION('ref_axis',(0.,0.,1.));
#139454=DIRECTION('center_axis',(1.,-3.49148133884313E-15,0.));
#139455=DIRECTION('ref_axis',(0.,0.,1.));
#139456=DIRECTION('center_axis',(1.,-3.49148133884313E-15,0.));
#139457=DIRECTION('ref_axis',(0.,0.,1.));
#139458=DIRECTION('center_axis',(1.,-3.49148133884313E-15,0.));
#139459=DIRECTION('ref_axis',(0.,0.,1.));
#139460=DIRECTION('center_axis',(1.,-3.49148133884313E-15,0.));
#139461=DIRECTION('ref_axis',(0.,0.,1.));
#139462=DIRECTION('center_axis',(1.,-3.49148133884313E-15,0.));
#139463=DIRECTION('ref_axis',(0.,0.,1.));
#139464=DIRECTION('center_axis',(1.,-3.49148133884313E-15,0.));
#139465=DIRECTION('ref_axis',(0.,0.,1.));
#139466=DIRECTION('center_axis',(1.,-3.49148133884313E-15,0.));
#139467=DIRECTION('ref_axis',(0.,0.,1.));
#139468=DIRECTION('center_axis',(1.,-3.49148133884313E-15,0.));
#139469=DIRECTION('ref_axis',(0.,0.,1.));
#139470=DIRECTION('center_axis',(1.,-3.49148133884313E-15,0.));
#139471=DIRECTION('ref_axis',(0.,0.,1.));
#139472=DIRECTION('center_axis',(-1.,3.49148133884313E-15,0.));
#139473=DIRECTION('ref_axis',(0.,0.,-1.));
#139474=DIRECTION('',(-3.02371153627746E-15,-0.866025403784438,0.500000000000001));
#139475=DIRECTION('',(-3.02371153627746E-15,-0.866025403784438,-0.500000000000001));
#139476=DIRECTION('',(0.,0.,-1.));
#139477=DIRECTION('',(3.02371153627745E-15,0.866025403784437,-0.500000000000003));
#139478=DIRECTION('',(3.02371153627745E-15,0.866025403784437,0.500000000000003));
#139479=DIRECTION('',(0.,0.,1.));
#139480=DIRECTION('center_axis',(-1.74574066942157E-15,-0.500000000000001,
0.866025403784438));
#139481=DIRECTION('ref_axis',(-3.02371153627746E-15,-0.866025403784438,
-0.500000000000001));
#139482=DIRECTION('',(1.,-3.49148133884313E-15,0.));
#139483=DIRECTION('',(1.,-3.49148133884313E-15,0.));
#139484=DIRECTION('center_axis',(-3.49148133884313E-15,-1.,0.));
#139485=DIRECTION('ref_axis',(0.,0.,-1.));
#139486=DIRECTION('',(1.,-3.49148133884313E-15,0.));
#139487=DIRECTION('center_axis',(-1.74574066942158E-15,-0.500000000000003,
-0.866025403784437));
#139488=DIRECTION('ref_axis',(3.02371153627745E-15,0.866025403784437,-0.500000000000003));
#139489=DIRECTION('',(1.,-3.49148133884313E-15,0.));
#139490=DIRECTION('center_axis',(1.74574066942158E-15,0.500000000000003,
-0.866025403784437));
#139491=DIRECTION('ref_axis',(3.02371153627745E-15,0.866025403784437,0.500000000000003));
#139492=DIRECTION('',(1.,-3.49148133884313E-15,0.));
#139493=DIRECTION('center_axis',(3.49148133884313E-15,1.,0.));
#139494=DIRECTION('ref_axis',(0.,0.,1.));
#139495=DIRECTION('',(1.,-3.49148133884313E-15,0.));
#139496=DIRECTION('center_axis',(1.74574066942157E-15,0.500000000000001,
0.866025403784438));
#139497=DIRECTION('ref_axis',(-3.02371153627746E-15,-0.866025403784438,
0.500000000000001));
#139498=DIRECTION('center_axis',(1.,-1.90843891001168E-31,-2.61618113230267E-16));
#139499=DIRECTION('ref_axis',(0.,1.,0.));
#139500=DIRECTION('center_axis',(0.,1.,0.));
#139501=DIRECTION('ref_axis',(-1.,0.,0.));
#139502=DIRECTION('',(0.,1.,0.));
#139503=DIRECTION('center_axis',(-3.57620498398977E-12,-1.,-7.43666695243917E-12));
#139504=DIRECTION('ref_axis',(-0.441622759424804,8.25151731278174E-12,-0.897200835018571));
#139505=DIRECTION('center_axis',(0.,1.,0.));
#139506=DIRECTION('ref_axis',(-1.,0.,0.));
#139507=DIRECTION('',(0.,1.,0.));
#139508=DIRECTION('center_axis',(0.,1.,0.));
#139509=DIRECTION('ref_axis',(-1.,0.,0.));
#139510=DIRECTION('',(0.,1.,0.));
#139511=DIRECTION('center_axis',(0.,1.,0.));
#139512=DIRECTION('ref_axis',(-1.,0.,0.));
#139513=DIRECTION('',(0.,1.,0.));
#139514=DIRECTION('center_axis',(0.,1.,0.));
#139515=DIRECTION('ref_axis',(-1.,0.,0.));
#139516=DIRECTION('',(0.,1.,0.));
#139517=DIRECTION('center_axis',(0.,1.,0.));
#139518=DIRECTION('ref_axis',(-1.,0.,0.));
#139519=DIRECTION('',(0.,1.,0.));
#139520=DIRECTION('center_axis',(0.,1.,1.4081690688991E-16));
#139521=DIRECTION('ref_axis',(1.40816906889911E-16,-1.4081690688991E-16,
1.));
#139522=DIRECTION('',(0.,-1.,-1.4081690688991E-16));
#139523=DIRECTION('center_axis',(0.,1.,1.4081690688991E-16));
#139524=DIRECTION('ref_axis',(1.40816906889911E-16,-1.4081690688991E-16,
1.));
#139525=DIRECTION('center_axis',(0.,1.,1.4081690688991E-16));
#139526=DIRECTION('ref_axis',(1.40816906889911E-16,-1.4081690688991E-16,
1.));
#139527=DIRECTION('',(0.,-1.,-1.4081690688991E-16));
#139528=DIRECTION('center_axis',(0.,1.,1.4081690688991E-16));
#139529=DIRECTION('ref_axis',(1.40816906889911E-16,-1.4081690688991E-16,
1.));
#139530=DIRECTION('center_axis',(0.,1.,1.4081690688991E-16));
#139531=DIRECTION('ref_axis',(1.40816906889911E-16,-1.4081690688991E-16,
1.));
#139532=DIRECTION('',(0.,-1.,-1.4081690688991E-16));
#139533=DIRECTION('center_axis',(0.,1.,1.4081690688991E-16));
#139534=DIRECTION('ref_axis',(1.40816906889911E-16,-1.4081690688991E-16,
1.));
#139535=DIRECTION('',(0.,-1.,-1.4081690688991E-16));
#139536=DIRECTION('center_axis',(0.,1.,1.4081690688991E-16));
#139537=DIRECTION('ref_axis',(1.40816906889911E-16,-1.4081690688991E-16,
1.));
#139538=DIRECTION('',(0.,-1.,-1.4081690688991E-16));
#139539=DIRECTION('center_axis',(0.,1.,1.4081690688991E-16));
#139540=DIRECTION('ref_axis',(1.40816906889911E-16,-1.4081690688991E-16,
1.));
#139541=DIRECTION('',(0.,-1.,-1.4081690688991E-16));
#139542=DIRECTION('center_axis',(0.,1.,1.4081690688991E-16));
#139543=DIRECTION('ref_axis',(1.40816906889911E-16,-1.4081690688991E-16,
1.));
#139544=DIRECTION('',(0.,-1.,-1.4081690688991E-16));
#139545=DIRECTION('center_axis',(0.,1.,1.4081690688991E-16));
#139546=DIRECTION('ref_axis',(1.40816906889911E-16,-1.4081690688991E-16,
1.));
#139547=DIRECTION('',(0.,-1.,-1.4081690688991E-16));
#139548=DIRECTION('center_axis',(0.,-1.,-1.4081690688991E-16));
#139549=DIRECTION('ref_axis',(-7.47361512810214E-16,-1.4081690688991E-16,
1.));
#139550=DIRECTION('center_axis',(0.,1.,1.4081690688991E-16));
#139551=DIRECTION('ref_axis',(1.40816906889911E-16,-1.4081690688991E-16,
1.));
#139552=DIRECTION('center_axis',(0.00785201424984197,0.999733823610251,
0.0216939577266995));
#139553=DIRECTION('ref_axis',(0.928088776890915,0.000790766293764068,-0.372358156749379));
#139554=DIRECTION('center_axis',(-7.68190179945114E-12,1.,1.1426270641458E-12));
#139555=DIRECTION('ref_axis',(0.141219054307676,-4.63451743285696E-14,0.989978372844804));
#139556=DIRECTION('center_axis',(-0.0191622393999958,-0.996432124380861,
-0.0821938567231223));
#139557=DIRECTION('ref_axis',(0.998980952014602,-0.0157214167558561,-0.0423071455807097));
#139558=DIRECTION('',(1.8616819539112E-16,-0.707106781186547,0.707106781186548));
#139559=DIRECTION('center_axis',(0.,-1.,-1.4081690688991E-16));
#139560=DIRECTION('ref_axis',(1.40816906889911E-16,-1.4081690688991E-16,
1.));
#139561=DIRECTION('center_axis',(0.,-1.,-1.4081690688991E-16));
#139562=DIRECTION('ref_axis',(-1.40816906889911E-16,1.40816906889911E-16,
-1.));
#139563=DIRECTION('center_axis',(0.,-1.,-1.4081690688991E-16));
#139564=DIRECTION('ref_axis',(-7.47361512810214E-16,-1.4081690688991E-16,
1.));
#139565=DIRECTION('center_axis',(0.0209809681760068,-0.99973153532607,-0.0098313909991016));
#139566=DIRECTION('ref_axis',(0.213430275538422,-0.00512812960618709,0.976944839676394));
#139567=DIRECTION('center_axis',(-0.0724020542557579,0.996321406376306,
0.0458431863627102));
#139568=DIRECTION('ref_axis',(0.528690912836516,-0.000636379508420693,0.848814180904875));
#139569=DIRECTION('center_axis',(0.,-1.,-1.4081690688991E-16));
#139570=DIRECTION('ref_axis',(-7.47361512810214E-16,-1.4081690688991E-16,
1.));
#139571=DIRECTION('',(-1.29769841440215E-17,0.707106781186545,-0.70710678118655));
#139572=DIRECTION('center_axis',(0.,1.,1.4081690688991E-16));
#139573=DIRECTION('ref_axis',(1.40816906889911E-16,-1.40816906889911E-16,
1.));
#139574=DIRECTION('center_axis',(0.,1.,1.4081690688991E-16));
#139575=DIRECTION('ref_axis',(1.40816906889911E-16,-1.4081690688991E-16,
1.));
#139576=DIRECTION('center_axis',(0.,1.,1.4081690688991E-16));
#139577=DIRECTION('ref_axis',(1.40816906889911E-16,-1.40816906889911E-16,
1.));
#139578=DIRECTION('center_axis',(0.,1.,1.4081690688991E-16));
#139579=DIRECTION('ref_axis',(1.40816906889911E-16,-1.40816906889911E-16,
1.));
#139580=DIRECTION('center_axis',(0.,1.,1.4081690688991E-16));
#139581=DIRECTION('ref_axis',(1.40816906889911E-16,-1.4081690688991E-16,
1.));
#139582=DIRECTION('center_axis',(0.,1.,1.4081690688991E-16));
#139583=DIRECTION('ref_axis',(1.40816906889911E-16,-1.4081690688991E-16,
1.));
#139584=DIRECTION('center_axis',(0.,1.,1.4081690688991E-16));
#139585=DIRECTION('ref_axis',(1.40816906889911E-16,-1.4081690688991E-16,
1.));
#139586=DIRECTION('center_axis',(0.,1.,1.4081690688991E-16));
#139587=DIRECTION('ref_axis',(1.40816906889911E-16,-1.4081690688991E-16,
1.));
#139588=DIRECTION('center_axis',(0.,1.,1.4081690688991E-16));
#139589=DIRECTION('ref_axis',(1.40816906889911E-16,-1.4081690688991E-16,
1.));
#139590=DIRECTION('center_axis',(0.,1.,1.4081690688991E-16));
#139591=DIRECTION('ref_axis',(1.40816906889911E-16,-1.4081690688991E-16,
1.));
#139592=DIRECTION('center_axis',(0.,1.,1.4081690688991E-16));
#139593=DIRECTION('ref_axis',(1.40816906889911E-16,-1.4081690688991E-16,
1.));
#139594=DIRECTION('center_axis',(0.,1.,1.4081690688991E-16));
#139595=DIRECTION('ref_axis',(1.40816906889911E-16,-1.4081690688991E-16,
1.));
#139596=DIRECTION('center_axis',(0.,1.,1.4081690688991E-16));
#139597=DIRECTION('ref_axis',(1.40816906889911E-16,-1.4081690688991E-16,
1.));
#139598=DIRECTION('center_axis',(0.,1.,1.4081690688991E-16));
#139599=DIRECTION('ref_axis',(1.40816906889911E-16,-1.4081690688991E-16,
1.));
#139600=DIRECTION('center_axis',(0.,1.,1.4081690688991E-16));
#139601=DIRECTION('ref_axis',(1.40816906889911E-16,-1.4081690688991E-16,
1.));
#139602=DIRECTION('center_axis',(0.,1.,1.4081690688991E-16));
#139603=DIRECTION('ref_axis',(1.40816906889911E-16,-1.4081690688991E-16,
1.));
#139604=DIRECTION('center_axis',(0.,-1.,-1.4081690688991E-16));
#139605=DIRECTION('ref_axis',(-1.40816906889911E-16,1.40816906889911E-16,
-1.));
#139606=DIRECTION('',(0.866025403784438,-7.04084534449553E-17,0.500000000000001));
#139607=DIRECTION('',(0.866025403784438,7.04084534449553E-17,-0.500000000000001));
#139608=DIRECTION('',(-1.40816906889911E-16,1.40816906889911E-16,-1.));
#139609=DIRECTION('',(-0.866025403784437,7.04084534449556E-17,-0.500000000000002));
#139610=DIRECTION('',(-0.866025403784437,-7.04084534449556E-17,0.500000000000003));
#139611=DIRECTION('',(1.40816906889911E-16,-1.40816906889911E-16,1.));
#139612=DIRECTION('center_axis',(0.500000000000001,-1.2195101864901E-16,
0.866025403784438));
#139613=DIRECTION('ref_axis',(0.866025403784438,7.04084534449554E-17,-0.500000000000001));
#139614=DIRECTION('',(0.,1.,1.40816906889911E-16));
#139615=DIRECTION('',(0.,1.,1.40816906889911E-16));
#139616=DIRECTION('center_axis',(1.,0.,-1.40816906889911E-16));
#139617=DIRECTION('ref_axis',(-1.40816906889911E-16,1.40816906889911E-16,
-1.));
#139618=DIRECTION('',(0.,1.,1.40816906889911E-16));
#139619=DIRECTION('center_axis',(0.500000000000002,1.2195101864901E-16,
-0.866025403784437));
#139620=DIRECTION('ref_axis',(-0.866025403784437,7.04084534449556E-17,-0.500000000000002));
#139621=DIRECTION('',(0.,1.,1.40816906889911E-16));
#139622=DIRECTION('center_axis',(-0.500000000000003,1.2195101864901E-16,
-0.866025403784437));
#139623=DIRECTION('ref_axis',(-0.866025403784437,-7.04084534449556E-17,
0.500000000000003));
#139624=DIRECTION('',(0.,1.,1.40816906889911E-16));
#139625=DIRECTION('center_axis',(-1.,0.,1.40816906889911E-16));
#139626=DIRECTION('ref_axis',(1.40816906889911E-16,-1.40816906889911E-16,
1.));
#139627=DIRECTION('',(0.,1.,1.40816906889911E-16));
#139628=DIRECTION('center_axis',(-0.500000000000001,-1.2195101864901E-16,
0.866025403784438));
#139629=DIRECTION('ref_axis',(0.866025403784438,-7.04084534449554E-17,0.500000000000001));
#139630=DIRECTION('center_axis',(0.,1.,0.));
#139631=DIRECTION('ref_axis',(-1.,0.,0.));
#139632=DIRECTION('center_axis',(0.,0.,-1.));
#139633=DIRECTION('ref_axis',(-1.,0.,0.));
#139634=DIRECTION('center_axis',(0.,0.,-1.));
#139635=DIRECTION('ref_axis',(-1.,0.,0.));
#139636=DIRECTION('',(0.642787609686534,-7.87187788734192E-17,-0.766044443118983));
#139637=DIRECTION('center_axis',(0.,0.,1.));
#139638=DIRECTION('ref_axis',(-1.,0.,0.));
#139639=DIRECTION('center_axis',(0.,0.,1.));
#139640=DIRECTION('ref_axis',(1.,0.,0.));
#139641=DIRECTION('center_axis',(0.,0.,1.));
#139642=DIRECTION('ref_axis',(1.,0.,0.));
#139643=DIRECTION('center_axis',(0.,0.,1.));
#139644=DIRECTION('ref_axis',(1.,0.,0.));
#139645=DIRECTION('',(-0.642787609686546,-7.87187788734207E-17,0.766044443118972));
#139646=DIRECTION('center_axis',(0.,0.,-1.));
#139647=DIRECTION('ref_axis',(1.,0.,0.));
#139648=DIRECTION('center_axis',(0.,0.,-1.));
#139649=DIRECTION('ref_axis',(-1.,0.,0.));
#139650=DIRECTION('center_axis',(0.,0.,-1.));
#139651=DIRECTION('ref_axis',(1.,0.,0.));
#139652=DIRECTION('',(-0.766044443118973,9.38133875270267E-17,0.642787609686545));
#139653=DIRECTION('center_axis',(0.,0.,1.));
#139654=DIRECTION('ref_axis',(1.,0.,0.));
#139655=DIRECTION('center_axis',(0.,0.,1.));
#139656=DIRECTION('ref_axis',(1.,0.,0.));
#139657=DIRECTION('center_axis',(0.,0.,1.));
#139658=DIRECTION('ref_axis',(-1.,0.,0.));
#139659=DIRECTION('center_axis',(0.,0.,1.));
#139660=DIRECTION('ref_axis',(-1.,0.,0.));
#139661=DIRECTION('',(0.766044443118977,9.38133875270271E-17,-0.642787609686541));
#139662=DIRECTION('center_axis',(0.,0.,-1.));
#139663=DIRECTION('ref_axis',(-1.,0.,0.));
#139664=DIRECTION('center_axis',(0.,0.,-1.));
#139665=DIRECTION('ref_axis',(-1.,0.,0.));
#139666=DIRECTION('',(0.,0.,1.));
#139667=DIRECTION('',(0.,0.,1.));
#139668=DIRECTION('center_axis',(0.,-1.,0.));
#139669=DIRECTION('ref_axis',(0.,0.,-1.));
#139670=DIRECTION('',(0.,-1.,0.));
#139671=DIRECTION('center_axis',(-1.,3.49148133884313E-15,0.));
#139672=DIRECTION('ref_axis',(0.,0.,-1.));
#139673=DIRECTION('',(-1.,3.49148133884313E-15,0.));
#139674=DIRECTION('center_axis',(0.,0.,-1.));
#139675=DIRECTION('ref_axis',(-1.,0.,0.));
#139676=DIRECTION('',(0.,0.,-1.));
#139677=DIRECTION('',(0.,0.,-1.));
#139678=DIRECTION('center_axis',(0.,0.,1.));
#139679=DIRECTION('ref_axis',(1.,0.,0.));
#139680=DIRECTION('center_axis',(0.,0.,-1.));
#139681=DIRECTION('ref_axis',(-1.,0.,0.));
#139682=DIRECTION('center_axis',(-1.4081690688991E-16,0.,-1.));
#139683=DIRECTION('ref_axis',(-1.,0.,1.4081690688991E-16));
#139684=DIRECTION('center_axis',(-1.4081690688991E-16,0.,-1.));
#139685=DIRECTION('ref_axis',(-1.,0.,1.4081690688991E-16));
#139686=DIRECTION('',(1.4081690688991E-16,0.,1.));
#139687=DIRECTION('center_axis',(0.,0.,-1.));
#139688=DIRECTION('ref_axis',(-1.,0.,0.));
#139689=DIRECTION('center_axis',(0.,0.,1.));
#139690=DIRECTION('ref_axis',(1.,0.,0.));
#139691=DIRECTION('center_axis',(-1.4081690688991E-16,0.,-1.));
#139692=DIRECTION('ref_axis',(-1.,0.,1.4081690688991E-16));
#139693=DIRECTION('',(0.,0.,1.));
#139694=DIRECTION('center_axis',(0.,0.,-1.));
#139695=DIRECTION('ref_axis',(-1.,0.,0.));
#139696=DIRECTION('center_axis',(0.,0.,-1.));
#139697=DIRECTION('ref_axis',(-1.,0.,0.));
#139698=DIRECTION('center_axis',(0.,0.,-1.));
#139699=DIRECTION('ref_axis',(-1.,0.,0.));
#139700=DIRECTION('center_axis',(1.22464679914735E-16,1.,0.));
#139701=DIRECTION('ref_axis',(1.,-1.22464679914735E-16,0.));
#139702=DIRECTION('center_axis',(0.,0.,1.));
#139703=DIRECTION('ref_axis',(-1.,0.,0.));
#139704=DIRECTION('center_axis',(0.,0.,1.));
#139705=DIRECTION('ref_axis',(-1.,0.,0.));
#139706=DIRECTION('center_axis',(0.,0.,1.));
#139707=DIRECTION('ref_axis',(1.,0.,0.));
#139708=DIRECTION('center_axis',(0.,0.,-1.));
#139709=DIRECTION('ref_axis',(-1.,0.,0.));
#139710=DIRECTION('',(0.,0.,1.));
#139711=DIRECTION('center_axis',(0.,0.,1.));
#139712=DIRECTION('ref_axis',(1.,0.,0.));
#139713=DIRECTION('center_axis',(0.,0.,-1.));
#139714=DIRECTION('ref_axis',(-1.,0.,0.));
#139715=DIRECTION('',(0.,0.,-1.));
#139716=DIRECTION('center_axis',(0.,0.,1.));
#139717=DIRECTION('ref_axis',(-1.,0.,0.));
#139718=DIRECTION('',(0.,0.,-1.));
#139719=DIRECTION('center_axis',(0.,0.,1.));
#139720=DIRECTION('ref_axis',(1.,0.,0.));
#139721=DIRECTION('center_axis',(0.,0.,-1.));
#139722=DIRECTION('ref_axis',(-1.,0.,0.));
#139723=DIRECTION('',(0.,0.,-1.));
#139724=DIRECTION('center_axis',(0.,0.,-1.));
#139725=DIRECTION('ref_axis',(-1.,0.,0.));
#139726=DIRECTION('center_axis',(0.,0.,-1.));
#139727=DIRECTION('ref_axis',(-1.,0.,0.));
#139728=DIRECTION('center_axis',(0.,0.,-1.));
#139729=DIRECTION('ref_axis',(-1.,0.,0.));
#139730=DIRECTION('',(0.,0.,-1.));
#139731=DIRECTION('center_axis',(0.,0.,-1.));
#139732=DIRECTION('ref_axis',(-1.,0.,0.));
#139733=DIRECTION('center_axis',(0.,0.,-1.));
#139734=DIRECTION('ref_axis',(-1.,0.,0.));
#139735=DIRECTION('center_axis',(0.,0.,-1.));
#139736=DIRECTION('ref_axis',(-1.,0.,0.));
#139737=DIRECTION('',(0.,0.,-1.));
#139738=DIRECTION('center_axis',(0.,0.,-1.));
#139739=DIRECTION('ref_axis',(-1.,0.,0.));
#139740=DIRECTION('center_axis',(0.,0.,-1.));
#139741=DIRECTION('ref_axis',(-1.,0.,0.));
#139742=DIRECTION('center_axis',(0.,0.,-1.));
#139743=DIRECTION('ref_axis',(-1.,0.,0.));
#139744=DIRECTION('',(0.,0.,-1.));
#139745=DIRECTION('center_axis',(0.,0.,-1.));
#139746=DIRECTION('ref_axis',(-1.,0.,0.));
#139747=DIRECTION('center_axis',(0.,0.,-1.));
#139748=DIRECTION('ref_axis',(-1.,0.,0.));
#139749=DIRECTION('center_axis',(0.,0.,-1.));
#139750=DIRECTION('ref_axis',(-1.,0.,0.));
#139751=DIRECTION('',(0.,0.,-1.));
#139752=DIRECTION('center_axis',(0.,0.,-1.));
#139753=DIRECTION('ref_axis',(-1.,0.,0.));
#139754=DIRECTION('center_axis',(0.,0.,-1.));
#139755=DIRECTION('ref_axis',(-1.,0.,0.));
#139756=DIRECTION('center_axis',(0.,0.,-1.));
#139757=DIRECTION('ref_axis',(-1.,0.,0.));
#139758=DIRECTION('',(0.,0.,-1.));
#139759=DIRECTION('center_axis',(0.,0.,-1.));
#139760=DIRECTION('ref_axis',(-1.,0.,0.));
#139761=DIRECTION('center_axis',(0.,0.,1.));
#139762=DIRECTION('ref_axis',(1.,0.,0.));
#139763=DIRECTION('center_axis',(0.,0.,-1.));
#139764=DIRECTION('ref_axis',(-1.,0.,0.));
#139765=DIRECTION('',(0.,0.,1.));
#139766=DIRECTION('center_axis',(0.,0.,-1.));
#139767=DIRECTION('ref_axis',(-1.,0.,0.));
#139768=DIRECTION('center_axis',(0.,0.,1.));
#139769=DIRECTION('ref_axis',(1.,0.,0.));
#139770=DIRECTION('center_axis',(0.,0.,-1.));
#139771=DIRECTION('ref_axis',(-1.,0.,0.));
#139772=DIRECTION('',(0.,0.,1.));
#139773=DIRECTION('center_axis',(0.,0.,-1.));
#139774=DIRECTION('ref_axis',(-1.,0.,0.));
#139775=DIRECTION('center_axis',(0.,0.,1.));
#139776=DIRECTION('ref_axis',(1.,0.,0.));
#139777=DIRECTION('center_axis',(0.,0.,-1.));
#139778=DIRECTION('ref_axis',(-1.,0.,0.));
#139779=DIRECTION('',(0.,0.,1.));
#139780=DIRECTION('center_axis',(0.,0.,-1.));
#139781=DIRECTION('ref_axis',(-1.,0.,0.));
#139782=DIRECTION('center_axis',(0.,0.,1.));
#139783=DIRECTION('ref_axis',(1.,0.,0.));
#139784=DIRECTION('center_axis',(0.,0.,-1.));
#139785=DIRECTION('ref_axis',(-1.,0.,0.));
#139786=DIRECTION('',(0.,0.,1.));
#139787=DIRECTION('center_axis',(0.,0.,-1.));
#139788=DIRECTION('ref_axis',(-1.,0.,0.));
#139789=DIRECTION('center_axis',(0.,0.,1.));
#139790=DIRECTION('ref_axis',(1.,0.,0.));
#139791=DIRECTION('',(0.,0.,1.));
#139792=DIRECTION('center_axis',(0.,0.,-1.));
#139793=DIRECTION('ref_axis',(-1.,0.,0.));
#139794=DIRECTION('',(0.,0.,1.));
#139795=DIRECTION('center_axis',(0.,0.,-1.));
#139796=DIRECTION('ref_axis',(-1.,0.,0.));
#139797=DIRECTION('center_axis',(1.,0.,0.));
#139798=DIRECTION('ref_axis',(0.,0.,-1.));
#139799=DIRECTION('',(0.,1.,0.));
#139800=DIRECTION('',(0.,0.,1.));
#139801=DIRECTION('',(0.,1.,0.));
#139802=DIRECTION('center_axis',(0.,0.,1.));
#139803=DIRECTION('ref_axis',(1.,0.,0.));
#139804=DIRECTION('center_axis',(0.,0.,-1.));
#139805=DIRECTION('ref_axis',(-1.,0.,0.));
#139806=DIRECTION('',(0.,0.,1.));
#139807=DIRECTION('center_axis',(0.,0.,-1.));
#139808=DIRECTION('ref_axis',(-1.,0.,0.));
#139809=DIRECTION('center_axis',(0.,-1.,0.));
#139810=DIRECTION('ref_axis',(0.,0.,-1.));
#139811=DIRECTION('',(1.,0.,0.));
#139812=DIRECTION('',(0.,0.,1.));
#139813=DIRECTION('',(1.,0.,0.));
#139814=DIRECTION('center_axis',(0.,0.,1.));
#139815=DIRECTION('ref_axis',(1.,0.,0.));
#139816=DIRECTION('center_axis',(0.,0.,-1.));
#139817=DIRECTION('ref_axis',(-1.,0.,0.));
#139818=DIRECTION('',(0.,0.,1.));
#139819=DIRECTION('center_axis',(0.,0.,-1.));
#139820=DIRECTION('ref_axis',(-1.,0.,0.));
#139821=DIRECTION('center_axis',(-1.,1.5419764230905E-16,0.));
#139822=DIRECTION('ref_axis',(-1.5419764230905E-16,-1.,0.));
#139823=DIRECTION('',(-1.5419764230905E-16,-1.,0.));
#139824=DIRECTION('',(0.,0.,1.));
#139825=DIRECTION('',(-1.5419764230905E-16,-1.,0.));
#139826=DIRECTION('center_axis',(0.,0.,1.));
#139827=DIRECTION('ref_axis',(1.,0.,0.));
#139828=DIRECTION('center_axis',(0.,0.,-1.));
#139829=DIRECTION('ref_axis',(-1.,0.,0.));
#139830=DIRECTION('',(0.,0.,1.));
#139831=DIRECTION('center_axis',(0.,0.,-1.));
#139832=DIRECTION('ref_axis',(-1.,0.,0.));
#139833=DIRECTION('center_axis',(0.,1.,0.));
#139834=DIRECTION('ref_axis',(0.,0.,1.));
#139835=DIRECTION('',(-1.,0.,0.));
#139836=DIRECTION('',(-1.,0.,0.));
#139837=DIRECTION('center_axis',(0.,0.,-1.));
#139838=DIRECTION('ref_axis',(-1.,0.,0.));
#139839=DIRECTION('',(0.,-1.,0.));
#139840=DIRECTION('center_axis',(0.,0.,1.));
#139841=DIRECTION('ref_axis',(-1.,0.,0.));
#139842=DIRECTION('',(1.,0.,0.));
#139843=DIRECTION('center_axis',(0.,0.,1.));
#139844=DIRECTION('ref_axis',(-1.,0.,0.));
#139845=DIRECTION('',(1.5419764230905E-16,1.,0.));
#139846=DIRECTION('center_axis',(0.,0.,1.));
#139847=DIRECTION('ref_axis',(-1.,0.,0.));
#139848=DIRECTION('',(-1.,0.,0.));
#139849=DIRECTION('center_axis',(0.,0.,1.));
#139850=DIRECTION('ref_axis',(-1.,0.,0.));
#139851=DIRECTION('center_axis',(0.,0.,-1.));
#139852=DIRECTION('ref_axis',(-1.,0.,0.));
#139853=DIRECTION('center_axis',(0.,0.,-1.));
#139854=DIRECTION('ref_axis',(-1.,0.,0.));
#139855=DIRECTION('center_axis',(0.,0.,-1.));
#139856=DIRECTION('ref_axis',(-1.,0.,0.));
#139857=DIRECTION('center_axis',(0.,0.,-1.));
#139858=DIRECTION('ref_axis',(-1.,0.,0.));
#139859=DIRECTION('center_axis',(0.,0.,-1.));
#139860=DIRECTION('ref_axis',(-1.,0.,0.));
#139861=DIRECTION('center_axis',(0.,0.,-1.));
#139862=DIRECTION('ref_axis',(-1.,0.,0.));
#139863=DIRECTION('',(1.,0.,0.));
#139864=DIRECTION('center_axis',(0.,0.,-1.));
#139865=DIRECTION('ref_axis',(-1.,0.,0.));
#139866=DIRECTION('',(0.,1.,0.));
#139867=DIRECTION('center_axis',(0.,0.,-1.));
#139868=DIRECTION('ref_axis',(-1.,0.,0.));
#139869=DIRECTION('',(-1.,0.,0.));
#139870=DIRECTION('center_axis',(0.,0.,-1.));
#139871=DIRECTION('ref_axis',(-1.,0.,0.));
#139872=DIRECTION('',(0.,-1.,0.));
#139873=DIRECTION('center_axis',(0.,0.,1.));
#139874=DIRECTION('ref_axis',(1.,0.,0.));
#139875=DIRECTION('',(0.,0.,1.));
#139876=DIRECTION('center_axis',(0.,0.,-1.));
#139877=DIRECTION('ref_axis',(-1.,0.,0.));
#139878=DIRECTION('',(0.,0.,1.));
#139879=DIRECTION('center_axis',(-1.,0.,0.));
#139880=DIRECTION('ref_axis',(0.,0.,1.));
#139881=DIRECTION('',(0.,0.,1.));
#139882=DIRECTION('',(1.5419764230905E-16,-1.,0.));
#139883=DIRECTION('center_axis',(0.,0.,1.));
#139884=DIRECTION('ref_axis',(1.,0.,0.));
#139885=DIRECTION('',(0.,0.,1.));
#139886=DIRECTION('center_axis',(0.,0.,-1.));
#139887=DIRECTION('ref_axis',(-1.,0.,0.));
#139888=DIRECTION('center_axis',(0.,1.,0.));
#139889=DIRECTION('ref_axis',(0.,0.,1.));
#139890=DIRECTION('',(0.,0.,1.));
#139891=DIRECTION('',(-1.,-1.5419764230905E-16,0.));
#139892=DIRECTION('center_axis',(0.,0.,1.));
#139893=DIRECTION('ref_axis',(1.,0.,0.));
#139894=DIRECTION('',(0.,0.,1.));
#139895=DIRECTION('center_axis',(0.,0.,-1.));
#139896=DIRECTION('ref_axis',(-1.,0.,0.));
#139897=DIRECTION('center_axis',(1.,0.,0.));
#139898=DIRECTION('ref_axis',(0.,0.,-1.));
#139899=DIRECTION('',(0.,0.,1.));
#139900=DIRECTION('',(0.,1.,0.));
#139901=DIRECTION('center_axis',(0.,0.,1.));
#139902=DIRECTION('ref_axis',(1.,0.,0.));
#139903=DIRECTION('',(0.,0.,1.));
#139904=DIRECTION('center_axis',(0.,0.,-1.));
#139905=DIRECTION('ref_axis',(-1.,0.,0.));
#139906=DIRECTION('center_axis',(0.,-1.,0.));
#139907=DIRECTION('ref_axis',(0.,0.,-1.));
#139908=DIRECTION('',(1.,0.,0.));
#139909=DIRECTION('center_axis',(0.,0.,-1.));
#139910=DIRECTION('ref_axis',(-1.,0.,0.));
#139911=DIRECTION('center_axis',(-1.,0.,0.));
#139912=DIRECTION('ref_axis',(0.,0.,1.));
#139913=DIRECTION('center_axis',(0.,-1.,0.));
#139914=DIRECTION('ref_axis',(0.,0.,-1.));
#139915=DIRECTION('center_axis',(-1.5419764230905E-16,-1.,0.));
#139916=DIRECTION('ref_axis',(1.,-1.5419764230905E-16,0.));
#139917=DIRECTION('center_axis',(0.,-1.,0.));
#139918=DIRECTION('ref_axis',(0.,0.,-1.));
#139919=DIRECTION('center_axis',(1.,0.,0.));
#139920=DIRECTION('ref_axis',(0.,0.,-1.));
#139921=DIRECTION('center_axis',(-1.,0.,0.));
#139922=DIRECTION('ref_axis',(0.,0.,1.));
#139923=DIRECTION('center_axis',(0.,0.,-1.));
#139924=DIRECTION('ref_axis',(-1.,0.,0.));
#139925=DIRECTION('center_axis',(-1.,0.,0.));
#139926=DIRECTION('ref_axis',(0.,0.,1.));
#139927=DIRECTION('center_axis',(0.,0.,-1.));
#139928=DIRECTION('ref_axis',(-1.,0.,0.));
#139929=DIRECTION('center_axis',(0.,-1.,0.));
#139930=DIRECTION('ref_axis',(0.,0.,-1.));
#139931=DIRECTION('center_axis',(-1.,0.,0.));
#139932=DIRECTION('ref_axis',(0.,0.,1.));
#139933=DIRECTION('center_axis',(-1.,0.,0.));
#139934=DIRECTION('ref_axis',(0.,0.,1.));
#139935=DIRECTION('center_axis',(0.,1.,0.));
#139936=DIRECTION('ref_axis',(0.,0.,1.));
#139937=DIRECTION('center_axis',(0.,-1.,0.));
#139938=DIRECTION('ref_axis',(0.,0.,-1.));
#139939=DIRECTION('center_axis',(0.,0.,-1.));
#139940=DIRECTION('ref_axis',(-1.,0.,0.));
#139941=DIRECTION('center_axis',(0.,0.,-1.));
#139942=DIRECTION('ref_axis',(-1.,0.,0.));
#139943=DIRECTION('center_axis',(0.,0.,1.));
#139944=DIRECTION('ref_axis',(-1.,-1.22464679914735E-16,0.));
#139945=DIRECTION('',(0.,0.,-1.));
#139946=DIRECTION('center_axis',(0.,0.,-1.));
#139947=DIRECTION('ref_axis',(-1.,0.,0.));
#139948=DIRECTION('',(0.,0.,-1.));
#139949=DIRECTION('center_axis',(0.,0.,1.));
#139950=DIRECTION('ref_axis',(-1.,0.,0.));
#139951=DIRECTION('center_axis',(0.,0.,-1.));
#139952=DIRECTION('ref_axis',(-1.,0.,0.));
#139953=DIRECTION('',(0.,-1.,0.));
#139954=DIRECTION('center_axis',(0.,0.,1.));
#139955=DIRECTION('ref_axis',(1.,0.,0.));
#139956=DIRECTION('',(1.00849943089951E-15,1.,0.));
#139957=DIRECTION('',(1.00849943089951E-15,-1.,0.));
#139958=DIRECTION('center_axis',(0.,0.,-1.));
#139959=DIRECTION('ref_axis',(1.,0.,0.));
#139960=DIRECTION('',(0.,1.,0.));
#139961=DIRECTION('center_axis',(0.,0.,-1.));
#139962=DIRECTION('ref_axis',(-1.,0.,0.));
#139963=DIRECTION('center_axis',(0.,0.,-1.));
#139964=DIRECTION('ref_axis',(-1.,0.,0.));
#139965=DIRECTION('center_axis',(-1.4081690688991E-16,0.,-1.));
#139966=DIRECTION('ref_axis',(-1.,0.,1.40816906889911E-16));
#139967=DIRECTION('center_axis',(0.,0.,-1.));
#139968=DIRECTION('ref_axis',(-1.,0.,0.));
#139969=DIRECTION('',(0.,0.,-1.));
#139970=DIRECTION('center_axis',(0.,0.,-1.));
#139971=DIRECTION('ref_axis',(1.,0.,0.));
#139972=DIRECTION('',(0.,0.,-1.));
#139973=DIRECTION('center_axis',(-1.,0.,0.));
#139974=DIRECTION('ref_axis',(0.,0.,1.));
#139975=DIRECTION('',(0.,1.,0.));
#139976=DIRECTION('center_axis',(1.,1.00849943089951E-15,0.));
#139977=DIRECTION('ref_axis',(-1.00849943089951E-15,1.,0.));
#139978=DIRECTION('',(1.00849943089951E-15,-1.,0.));
#139979=DIRECTION('center_axis',(0.,0.,1.));
#139980=DIRECTION('ref_axis',(1.,0.,0.));
#139981=DIRECTION('',(1.00849943089951E-15,1.,0.));
#139982=DIRECTION('center_axis',(0.,0.,1.));
#139983=DIRECTION('ref_axis',(1.,0.,0.));
#139984=DIRECTION('',(0.,-1.,0.));
#139985=DIRECTION('center_axis',(0.,0.,-1.));
#139986=DIRECTION('ref_axis',(-1.,0.,0.));
#139987=DIRECTION('',(0.,0.,-1.));
#139988=DIRECTION('',(0.,0.,-1.));
#139989=DIRECTION('center_axis',(-1.,0.,0.));
#139990=DIRECTION('ref_axis',(0.,0.,1.));
#139991=DIRECTION('center_axis',(1.,-1.00849943089951E-15,0.));
#139992=DIRECTION('ref_axis',(-1.00849943089951E-15,-1.,0.));
#167144=CARTESIAN_POINT('',(0.,0.,0.));
#167145=CARTESIAN_POINT('Origin',(0.,88.06196,30.1625));
#167146=CARTESIAN_POINT('',(-2.19545458095144E-14,88.8392,27.2224678294277));
#167147=CARTESIAN_POINT('Origin',(0.,88.8392,30.1625));
#167148=CARTESIAN_POINT('',(4.63595923051442E-16,86.5786,26.3769520087407));
#167149=CARTESIAN_POINT('Origin',(-5.27423947715602E-16,88.06196,25.8557566346246));
#167150=CARTESIAN_POINT('',(-4.63595923051442E-16,86.5786,33.9480479912593));
#167151=CARTESIAN_POINT('Origin',(0.,86.5786,30.1625));
#167152=CARTESIAN_POINT('Origin',(0.,86.5786,30.1625));
#167153=CARTESIAN_POINT('Origin',(8.67361737988404E-16,85.9309,24.3332830071269));
#167154=CARTESIAN_POINT('',(0.253999999997468,85.5163328910991,23.893342102003));
#167155=CARTESIAN_POINT('',(-0.254,85.5163328910999,23.8933421020044));
#167156=CARTESIAN_POINT('Ctrl Pts',(-0.253999999999999,85.5163328910999,
23.8933421020044));
#167157=CARTESIAN_POINT('Ctrl Pts',(-0.239161970832706,85.5117377397736,
23.8847753618705));
#167158=CARTESIAN_POINT('Ctrl Pts',(-0.223780545620189,85.5075216342437,
23.876898996833));
#167159=CARTESIAN_POINT('Ctrl Pts',(-0.142699715976584,85.4880734540668,
23.8405156203159));
#167160=CARTESIAN_POINT('Ctrl Pts',(-0.0697029152864557,85.4800084964366,
23.8252830071269));
#167161=CARTESIAN_POINT('Ctrl Pts',(0.0697029152864574,85.4800084964366,
23.8252830071269));
#167162=CARTESIAN_POINT('Ctrl Pts',(0.142699715976585,85.4880734540668,
23.8405156203159));
#167163=CARTESIAN_POINT('Ctrl Pts',(0.223780545619289,85.5075216342435,
23.8768989968326));
#167164=CARTESIAN_POINT('Ctrl Pts',(0.239161970830955,85.5117377397731,
23.8847753618696));
#167165=CARTESIAN_POINT('Ctrl Pts',(0.253999999997466,85.5163328910991,
23.893342102003));
#167166=CARTESIAN_POINT('',(0.254,82.4084671089001,23.8933421020044));
#167167=CARTESIAN_POINT('',(0.254000000000001,85.9309,23.8933421020044));
#167168=CARTESIAN_POINT('',(-0.253999999997468,82.4084671089009,23.893342102003));
#167169=CARTESIAN_POINT('Ctrl Pts',(0.254000000000002,82.4084671089001,
23.8933421020044));
#167170=CARTESIAN_POINT('Ctrl Pts',(0.23916197083271,82.4130622602264,23.8847753618705));
#167171=CARTESIAN_POINT('Ctrl Pts',(0.223780545620191,82.4172783657563,
23.876898996833));
#167172=CARTESIAN_POINT('Ctrl Pts',(0.142699715976589,82.4367265459332,
23.8405156203159));
#167173=CARTESIAN_POINT('Ctrl Pts',(0.0697029152864575,82.4447915035635,
23.8252830071269));
#167174=CARTESIAN_POINT('Ctrl Pts',(-0.0697029152864557,82.4447915035635,
23.8252830071269));
#167175=CARTESIAN_POINT('Ctrl Pts',(-0.142699715976587,82.4367265459332,
23.8405156203159));
#167176=CARTESIAN_POINT('Ctrl Pts',(-0.223780545619291,82.4172783657565,
23.8768989968326));
#167177=CARTESIAN_POINT('Ctrl Pts',(-0.239161970830955,82.4130622602269,
23.8847753618696));
#167178=CARTESIAN_POINT('Ctrl Pts',(-0.253999999997466,82.4084671089009,
23.893342102003));
#167179=CARTESIAN_POINT('',(-0.254,85.9309,23.8933421020044));
#167180=CARTESIAN_POINT('Origin',(0.,81.9939,30.1625));
#167181=CARTESIAN_POINT('',(-2.778125,81.9939,25.3506463502227));
#167182=CARTESIAN_POINT('',(2.778125,81.9939,25.3506463502227));
#167183=CARTESIAN_POINT('Origin',(0.,81.9939,30.1625));
#167184=CARTESIAN_POINT('Ctrl Pts',(-0.253999999996936,82.4084671089011,
23.8933421020027));
#167185=CARTESIAN_POINT('Ctrl Pts',(-1.59266295510872,81.9939,24.6662195194906));
#167186=CARTESIAN_POINT('Ctrl Pts',(-2.778125,81.9939,25.3506463502227));
#167187=CARTESIAN_POINT('Ctrl Pts',(2.77812500000002,81.9939,25.3506463502227));
#167188=CARTESIAN_POINT('Ctrl Pts',(1.59266295510979,81.9939,24.6662195194913));
#167189=CARTESIAN_POINT('Ctrl Pts',(0.253999999999473,82.4084671089003,
23.8933421020041));
#167190=CARTESIAN_POINT('Origin',(0.,92.3825,30.1625));
#167191=CARTESIAN_POINT('',(-6.29897081141441E-16,81.9939,25.019));
#167192=CARTESIAN_POINT('Origin',(0.,81.9939,30.1625));
#167193=CARTESIAN_POINT('',(-6.29897081141441E-16,76.444,25.019));
#167194=CARTESIAN_POINT('',(-6.29897081141441E-16,92.3825,25.019));
#167195=CARTESIAN_POINT('Origin',(0.,76.444,30.1625));
#167196=CARTESIAN_POINT('Origin',(0.,85.9309,30.1625));
#167197=CARTESIAN_POINT('',(-2.778125,85.9309,34.9743536497773));
#167198=CARTESIAN_POINT('',(-6.80444377776248E-16,85.9309,35.71875));
#167199=CARTESIAN_POINT('Origin',(0.,85.9309,30.1625));
#167200=CARTESIAN_POINT('',(-0.25399999999747,85.5163328910991,36.431657897997));
#167201=CARTESIAN_POINT('Ctrl Pts',(-0.253999999996926,85.5163328910989,
36.4316578979973));
#167202=CARTESIAN_POINT('Ctrl Pts',(-1.59266295510872,85.9309,35.6587804805094));
#167203=CARTESIAN_POINT('Ctrl Pts',(-2.77812499999999,85.9309,34.9743536497773));
#167204=CARTESIAN_POINT('',(0.253999999999998,85.5163328910999,36.4316578979955));
#167205=CARTESIAN_POINT('Ctrl Pts',(-0.253999999997471,85.5163328910991,
36.431657897997));
#167206=CARTESIAN_POINT('Ctrl Pts',(-0.239161970830961,85.5117377397731,
36.4402246381304));
#167207=CARTESIAN_POINT('Ctrl Pts',(-0.22378054561929,85.5075216342435,
36.4481010031674));
#167208=CARTESIAN_POINT('Ctrl Pts',(-0.142699715976586,85.4880734540668,
36.4844843796841));
#167209=CARTESIAN_POINT('Ctrl Pts',(-0.0697029152864572,85.4800084964366,
36.4997169928731));
#167210=CARTESIAN_POINT('Ctrl Pts',(0.0697029152864559,85.4800084964366,
36.4997169928731));
#167211=CARTESIAN_POINT('Ctrl Pts',(0.142699715976579,85.4880734540668,
36.4844843796841));
#167212=CARTESIAN_POINT('Ctrl Pts',(0.223780545620182,85.5075216342437,
36.448101003167));
#167213=CARTESIAN_POINT('Ctrl Pts',(0.239161970832703,85.5117377397736,
36.4402246381295));
#167214=CARTESIAN_POINT('Ctrl Pts',(0.253999999999996,85.5163328910999,
36.4316578979955));
#167215=CARTESIAN_POINT('',(2.778125,85.9309,34.9743536497773));
#167216=CARTESIAN_POINT('Ctrl Pts',(2.77812499999997,85.9309,34.9743536497773));
#167217=CARTESIAN_POINT('Ctrl Pts',(1.59266295510976,85.9309,35.6587804805088));
#167218=CARTESIAN_POINT('Ctrl Pts',(0.253999999999462,85.5163328910997,
36.4316578979959));
#167219=CARTESIAN_POINT('Origin',(0.,85.9309,30.1625));
#167220=CARTESIAN_POINT('Origin',(0.,86.5786,30.1625));
#167221=CARTESIAN_POINT('',(2.778125,85.9309,25.3506463502227));
#167222=CARTESIAN_POINT('',(-2.778125,85.9309,25.3506463502227));
#167223=CARTESIAN_POINT('Origin',(0.,85.9309,30.1625));
#167224=CARTESIAN_POINT('',(-5.55625,85.9309,30.1625));
#167225=CARTESIAN_POINT('Origin',(0.,85.9309,30.1625));
#167226=CARTESIAN_POINT('Origin',(0.,85.9309,30.1625));
#167227=CARTESIAN_POINT('',(-4.63595923051442E-16,86.5786,33.9480479912593));
#167228=CARTESIAN_POINT('',(5.55625,85.9309,30.1625));
#167229=CARTESIAN_POINT('Origin',(0.,85.9309,30.1625));
#167230=CARTESIAN_POINT('Origin',(0.,85.9309,30.1625));
#167231=CARTESIAN_POINT('Origin',(0.,90.50036,30.1625));
#167232=CARTESIAN_POINT('',(4.10011707243361E-16,90.0597468392398,26.8145003356982));
#167233=CARTESIAN_POINT('Origin',(0.,90.0597468392398,30.1625));
#167234=CARTESIAN_POINT('Origin',(0.,90.1426015156173,30.1625));
#167235=CARTESIAN_POINT('',(4.05855902421057E-16,90.3626969268466,33.4765649426727));
#167236=CARTESIAN_POINT('',(-4.05855902421057E-16,90.3626969268466,26.8484350573273));
#167237=CARTESIAN_POINT('Origin',(0.,90.3626969268466,30.1625));
#167238=CARTESIAN_POINT('Origin',(0.,90.3626969268466,30.1625));
#167239=CARTESIAN_POINT('Origin',(-3.32911451644902E-16,90.1426015156173,
27.4440716998837));
#167240=CARTESIAN_POINT('Origin',(0.,92.8100477056147,30.1625));
#167241=CARTESIAN_POINT('',(-2.95107708105312E-16,92.8100477056147,32.5722373080204));
#167242=CARTESIAN_POINT('',(-2.95107708105312E-16,92.8100477056147,32.5722373080204));
#167243=CARTESIAN_POINT('',(2.95107708105313E-16,92.8100477056147,27.7527626919796));
#167244=CARTESIAN_POINT('Origin',(0.,92.8100477056147,30.1625));
#167245=CARTESIAN_POINT('Origin',(0.,92.8100477056147,30.1625));
#167246=CARTESIAN_POINT('Origin',(0.,92.7,30.1625));
#167247=CARTESIAN_POINT('',(-2.58635482717236E-16,93.0175,28.0505810132578));
#167248=CARTESIAN_POINT('Origin',(0.,93.0175,30.1625));
#167249=CARTESIAN_POINT('Origin',(-2.58635482717236E-16,92.7,28.0505810132578));
#167250=CARTESIAN_POINT('Origin',(0.,92.3825,30.1625));
#167251=CARTESIAN_POINT('',(-1.16647607618785E-16,92.3825,29.21));
#167252=CARTESIAN_POINT('Origin',(0.,92.3825,30.1625));
#167253=CARTESIAN_POINT('',(-1.16647607618785E-16,93.0175,29.21));
#167254=CARTESIAN_POINT('',(-1.16647607618785E-16,92.3825,29.21));
#167255=CARTESIAN_POINT('Origin',(0.,93.0175,30.1625));
#167256=CARTESIAN_POINT('Origin',(-6.65127195049617E-15,93.0175,29.21));
#167257=CARTESIAN_POINT('Origin',(-6.65127195049617E-15,92.3825,29.21));
#167258=CARTESIAN_POINT('Origin',(0.,85.9309,30.1625));
#167259=CARTESIAN_POINT('Ctrl Pts',(0.253999999996886,85.5163328910989,
23.8933421020026));
#167260=CARTESIAN_POINT('Ctrl Pts',(1.5926629551087,85.9309,24.6662195194906));
#167261=CARTESIAN_POINT('Ctrl Pts',(2.77812499999999,85.9309,25.3506463502227));
#167262=CARTESIAN_POINT('Ctrl Pts',(-2.77812500000002,85.9309,25.3506463502227));
#167263=CARTESIAN_POINT('Ctrl Pts',(-1.59266295510979,85.9309,24.6662195194913));
#167264=CARTESIAN_POINT('Ctrl Pts',(-0.253999999999478,85.5163328910998,
23.8933421020042));
#167265=CARTESIAN_POINT('Origin',(0.,85.9309,30.1625));
#167266=CARTESIAN_POINT('',(5.55625,85.5163328910998,27.2478915035631));
#167267=CARTESIAN_POINT('Ctrl Pts',(5.55625,85.5163328910997,27.2478915035625));
#167268=CARTESIAN_POINT('Ctrl Pts',(5.55625,85.9309,28.7936463385369));
#167269=CARTESIAN_POINT('Ctrl Pts',(5.55625,85.9309,30.1625));
#167270=CARTESIAN_POINT('',(5.30225,85.5163328910999,26.807950598441));
#167271=CARTESIAN_POINT('Ctrl Pts',(5.55625,85.5163328910998,27.2478915035631));
#167272=CARTESIAN_POINT('Ctrl Pts',(5.55624999999999,85.5117377397735,27.2307580232952));
#167273=CARTESIAN_POINT('Ctrl Pts',(5.55538041960567,85.5075216342437,27.2134991357962));
#167274=CARTESIAN_POINT('Ctrl Pts',(5.54634893312311,85.4880734540669,27.1250893893065));
#167275=CARTESIAN_POINT('Ctrl Pts',(5.52304236276573,85.4800084964366,27.0542559989194));
#167276=CARTESIAN_POINT('Ctrl Pts',(5.45333944747927,85.4800084964365,26.9335270082076));
#167277=CARTESIAN_POINT('Ctrl Pts',(5.40364921714652,85.4880734540669,26.8779262310094));
#167278=CARTESIAN_POINT('Ctrl Pts',(5.3315998739855,85.5075216342438,26.8258998610367));
#167279=CARTESIAN_POINT('Ctrl Pts',(5.31708802916729,85.5117377397736,26.816517338575));
#167280=CARTESIAN_POINT('Ctrl Pts',(5.30225,85.5163328910999,26.807950598441));
#167281=CARTESIAN_POINT('Ctrl Pts',(2.77812499999999,85.9309,25.3506463502227));
#167282=CARTESIAN_POINT('Ctrl Pts',(3.96358704489022,85.9309,26.0350731809542));
#167283=CARTESIAN_POINT('Ctrl Pts',(5.30225000000053,85.5163328910998,26.8079505984413));
#167284=CARTESIAN_POINT('Origin',(0.,85.9309,30.1625));
#167285=CARTESIAN_POINT('',(5.30225000000253,85.5163328910991,33.5170494015576));
#167286=CARTESIAN_POINT('Ctrl Pts',(5.30225000000307,85.5163328910989,33.5170494015572));
#167287=CARTESIAN_POINT('Ctrl Pts',(3.96358704489126,85.9309,34.2899268190452));
#167288=CARTESIAN_POINT('Ctrl Pts',(2.77812499999997,85.9309,34.9743536497773));
#167289=CARTESIAN_POINT('',(5.55625,85.5163328910999,33.0771084964365));
#167290=CARTESIAN_POINT('Ctrl Pts',(5.30225000000253,85.5163328910991,33.5170494015576));
#167291=CARTESIAN_POINT('Ctrl Pts',(5.31708802916894,85.5117377397731,33.508482661424));
#167292=CARTESIAN_POINT('Ctrl Pts',(5.33159987398629,85.5075216342435,33.4991001389628));
#167293=CARTESIAN_POINT('Ctrl Pts',(5.40364921714653,85.4880734540669,33.4470737689906));
#167294=CARTESIAN_POINT('Ctrl Pts',(5.45333944747927,85.4800084964366,33.3914729917924));
#167295=CARTESIAN_POINT('Ctrl Pts',(5.52304236276573,85.4800084964366,33.2707440010806));
#167296=CARTESIAN_POINT('Ctrl Pts',(5.54634893312311,85.4880734540668,33.1999106106935));
#167297=CARTESIAN_POINT('Ctrl Pts',(5.55538041960568,85.5075216342437,33.1115008642037));
#167298=CARTESIAN_POINT('Ctrl Pts',(5.55625,85.5117377397736,33.0942419767045));
#167299=CARTESIAN_POINT('Ctrl Pts',(5.55625,85.5163328910999,33.0771084964365));
#167300=CARTESIAN_POINT('Ctrl Pts',(5.55625,85.9309,30.1625));
#167301=CARTESIAN_POINT('Ctrl Pts',(5.55625,85.9309,31.5313536614629));
#167302=CARTESIAN_POINT('Ctrl Pts',(5.55625,85.5163328910997,33.0771084964371));
#167303=CARTESIAN_POINT('Origin',(0.,85.9309,30.1625));
#167304=CARTESIAN_POINT('',(-5.55625,85.5163328910999,33.0771084964365));
#167305=CARTESIAN_POINT('Ctrl Pts',(-5.55625,85.5163328910998,33.0771084964371));
#167306=CARTESIAN_POINT('Ctrl Pts',(-5.55625,85.9309000000001,31.5313536614629));
#167307=CARTESIAN_POINT('Ctrl Pts',(-5.55625,85.9309000000001,30.1625));
#167308=CARTESIAN_POINT('',(-5.30225,85.5163328910999,33.517049401559));
#167309=CARTESIAN_POINT('Ctrl Pts',(-5.55625,85.5163328910999,33.0771084964365));
#167310=CARTESIAN_POINT('Ctrl Pts',(-5.55625,85.5117377397736,33.0942419767045));
#167311=CARTESIAN_POINT('Ctrl Pts',(-5.55538041960568,85.5075216342438,
33.1115008642037));
#167312=CARTESIAN_POINT('Ctrl Pts',(-5.54634893312311,85.4880734540669,
33.1999106106935));
#167313=CARTESIAN_POINT('Ctrl Pts',(-5.52304236276573,85.4800084964366,
33.2707440010806));
#167314=CARTESIAN_POINT('Ctrl Pts',(-5.45333944747927,85.4800084964366,
33.3914729917924));
#167315=CARTESIAN_POINT('Ctrl Pts',(-5.40364921714652,85.4880734540669,
33.4470737689906));
#167316=CARTESIAN_POINT('Ctrl Pts',(-5.33159987398549,85.5075216342438,
33.4991001389633));
#167317=CARTESIAN_POINT('Ctrl Pts',(-5.31708802916729,85.5117377397736,
33.5084826614251));
#167318=CARTESIAN_POINT('Ctrl Pts',(-5.30225,85.5163328910999,33.517049401559));
#167319=CARTESIAN_POINT('Ctrl Pts',(-2.77812499999999,85.9309,34.9743536497773));
#167320=CARTESIAN_POINT('Ctrl Pts',(-3.96358704489021,85.9309,34.2899268190458));
#167321=CARTESIAN_POINT('Ctrl Pts',(-5.30225000000052,85.5163328910997,
33.5170494015587));
#167322=CARTESIAN_POINT('Origin',(0.,85.9309,30.1625));
#167323=CARTESIAN_POINT('',(-5.30225000000253,85.5163328910991,26.8079505984424));
#167324=CARTESIAN_POINT('Ctrl Pts',(-5.30225000000299,85.516332891099,26.8079505984427));
#167325=CARTESIAN_POINT('Ctrl Pts',(-3.96358704489126,85.9309,26.0350731809548));
#167326=CARTESIAN_POINT('Ctrl Pts',(-2.77812500000002,85.9309,25.3506463502227));
#167327=CARTESIAN_POINT('',(-5.55625,85.5163328910998,27.2478915035631));
#167328=CARTESIAN_POINT('Ctrl Pts',(-5.30225000000253,85.5163328910991,
26.8079505984424));
#167329=CARTESIAN_POINT('Ctrl Pts',(-5.31708802916895,85.5117377397731,
26.816517338576));
#167330=CARTESIAN_POINT('Ctrl Pts',(-5.3315998739863,85.5075216342435,26.8258998610372));
#167331=CARTESIAN_POINT('Ctrl Pts',(-5.40364921714653,85.4880734540668,
26.8779262310094));
#167332=CARTESIAN_POINT('Ctrl Pts',(-5.45333944747927,85.4800084964366,
26.9335270082076));
#167333=CARTESIAN_POINT('Ctrl Pts',(-5.52304236276573,85.4800084964366,
27.0542559989194));
#167334=CARTESIAN_POINT('Ctrl Pts',(-5.54634893312311,85.4880734540668,
27.1250893893065));
#167335=CARTESIAN_POINT('Ctrl Pts',(-5.55538041960567,85.5075216342437,
27.2134991357962));
#167336=CARTESIAN_POINT('Ctrl Pts',(-5.55624999999999,85.5117377397735,
27.2307580232952));
#167337=CARTESIAN_POINT('Ctrl Pts',(-5.55625,85.5163328910998,27.2478915035631));
#167338=CARTESIAN_POINT('Ctrl Pts',(-5.55625,85.9309000000001,30.1625));
#167339=CARTESIAN_POINT('Ctrl Pts',(-5.55625,85.9309000000001,28.7936463385369));
#167340=CARTESIAN_POINT('Ctrl Pts',(-5.55625,85.5163328910997,27.2478915035624));
#167341=CARTESIAN_POINT('Origin',(-3.59168685326793E-14,76.444,25.019));
#167342=CARTESIAN_POINT('Origin',(-3.87990863778943E-14,81.9939,24.60625));
#167343=CARTESIAN_POINT('',(5.55625,81.9939,30.1625));
#167344=CARTESIAN_POINT('Origin',(0.,81.9939,30.1625));
#167345=CARTESIAN_POINT('',(2.778125,81.9939,34.9743536497773));
#167346=CARTESIAN_POINT('Origin',(0.,81.9939,30.1625));
#167347=CARTESIAN_POINT('',(-2.778125,81.9939,34.9743536497773));
#167348=CARTESIAN_POINT('Origin',(0.,81.9939,30.1625));
#167349=CARTESIAN_POINT('',(-5.55625,81.9939,30.1625));
#167350=CARTESIAN_POINT('Origin',(0.,81.9939,30.1625));
#167351=CARTESIAN_POINT('Origin',(0.,81.9939,30.1625));
#167352=CARTESIAN_POINT('Origin',(0.,81.9939,30.1625));
#167353=CARTESIAN_POINT('',(-5.55625,82.4084671089002,27.2478915035631));
#167354=CARTESIAN_POINT('Ctrl Pts',(-5.55625,82.4084671089004,27.2478915035625));
#167355=CARTESIAN_POINT('Ctrl Pts',(-5.55625,81.9939,28.793646338537));
#167356=CARTESIAN_POINT('Ctrl Pts',(-5.55625,81.9939,30.1625000000001));
#167357=CARTESIAN_POINT('',(-5.30225,82.4084671089001,26.807950598441));
#167358=CARTESIAN_POINT('Ctrl Pts',(-5.55625,82.4084671089002,27.2478915035631));
#167359=CARTESIAN_POINT('Ctrl Pts',(-5.55624999999999,82.4130622602265,
27.2307580232952));
#167360=CARTESIAN_POINT('Ctrl Pts',(-5.55538041960567,82.4172783657563,
27.2134991357962));
#167361=CARTESIAN_POINT('Ctrl Pts',(-5.54634893312311,82.4367265459332,
27.1250893893065));
#167362=CARTESIAN_POINT('Ctrl Pts',(-5.52304236276573,82.4447915035635,
27.0542559989194));
#167363=CARTESIAN_POINT('Ctrl Pts',(-5.45333944747927,82.4447915035635,
26.9335270082076));
#167364=CARTESIAN_POINT('Ctrl Pts',(-5.40364921714653,82.4367265459332,
26.8779262310094));
#167365=CARTESIAN_POINT('Ctrl Pts',(-5.3315998739855,82.4172783657563,26.8258998610367));
#167366=CARTESIAN_POINT('Ctrl Pts',(-5.3170880291673,82.4130622602264,26.816517338575));
#167367=CARTESIAN_POINT('Ctrl Pts',(-5.30225000000001,82.4084671089001,
26.807950598441));
#167368=CARTESIAN_POINT('Ctrl Pts',(-2.77812500000003,81.9939,25.3506463502227));
#167369=CARTESIAN_POINT('Ctrl Pts',(-3.96358704489024,81.9939,26.0350731809542));
#167370=CARTESIAN_POINT('Ctrl Pts',(-5.30225000000053,82.4084671089003,
26.8079505984413));
#167371=CARTESIAN_POINT('Origin',(0.,81.9939,30.1625));
#167372=CARTESIAN_POINT('',(-5.30225000000254,82.4084671089009,33.5170494015576));
#167373=CARTESIAN_POINT('Ctrl Pts',(-5.30225000000307,82.4084671089011,
33.5170494015573));
#167374=CARTESIAN_POINT('Ctrl Pts',(-3.96358704489128,81.9939,34.2899268190452));
#167375=CARTESIAN_POINT('Ctrl Pts',(-2.778125,81.9939,34.9743536497773));
#167376=CARTESIAN_POINT('',(-5.55625,82.4084671089001,33.0771084964365));
#167377=CARTESIAN_POINT('Ctrl Pts',(-5.30225000000254,82.4084671089009,
33.5170494015576));
#167378=CARTESIAN_POINT('Ctrl Pts',(-5.31708802916895,82.4130622602269,
33.508482661424));
#167379=CARTESIAN_POINT('Ctrl Pts',(-5.33159987398629,82.4172783657565,
33.4991001389628));
#167380=CARTESIAN_POINT('Ctrl Pts',(-5.40364921714652,82.4367265459332,
33.4470737689906));
#167381=CARTESIAN_POINT('Ctrl Pts',(-5.45333944747927,82.4447915035635,
33.3914729917924));
#167382=CARTESIAN_POINT('Ctrl Pts',(-5.52304236276573,82.4447915035635,
33.2707440010806));
#167383=CARTESIAN_POINT('Ctrl Pts',(-5.54634893312311,82.4367265459332,
33.1999106106935));
#167384=CARTESIAN_POINT('Ctrl Pts',(-5.55538041960568,82.4172783657563,
33.1115008642037));
#167385=CARTESIAN_POINT('Ctrl Pts',(-5.55625,82.4130622602264,33.0942419767045));
#167386=CARTESIAN_POINT('Ctrl Pts',(-5.55625,82.4084671089001,33.0771084964365));
#167387=CARTESIAN_POINT('Ctrl Pts',(-5.55625,81.9939,30.1625000000001));
#167388=CARTESIAN_POINT('Ctrl Pts',(-5.55625,81.9939,31.531353661463));
#167389=CARTESIAN_POINT('Ctrl Pts',(-5.55625,82.4084671089003,33.0771084964372));
#167390=CARTESIAN_POINT('Origin',(0.,81.9939,30.1625));
#167391=CARTESIAN_POINT('',(0.253999999997469,82.4084671089009,36.431657897997));
#167392=CARTESIAN_POINT('Ctrl Pts',(0.253999999996946,82.4084671089011,
36.4316578979973));
#167393=CARTESIAN_POINT('Ctrl Pts',(1.59266295510873,81.9939,35.6587804805093));
#167394=CARTESIAN_POINT('Ctrl Pts',(2.77812500000001,81.9939,34.9743536497773));
#167395=CARTESIAN_POINT('',(-0.253999999999999,82.4084671089001,36.4316578979955));
#167396=CARTESIAN_POINT('Ctrl Pts',(0.253999999997469,82.4084671089009,
36.431657897997));
#167397=CARTESIAN_POINT('Ctrl Pts',(0.239161970830958,82.4130622602269,
36.4402246381304));
#167398=CARTESIAN_POINT('Ctrl Pts',(0.22378054561929,82.4172783657565,36.4481010031674));
#167399=CARTESIAN_POINT('Ctrl Pts',(0.142699715976588,82.4367265459332,
36.4844843796841));
#167400=CARTESIAN_POINT('Ctrl Pts',(0.0697029152864558,82.4447915035635,
36.4997169928731));
#167401=CARTESIAN_POINT('Ctrl Pts',(-0.0697029152864573,82.4447915035635,
36.4997169928731));
#167402=CARTESIAN_POINT('Ctrl Pts',(-0.142699715976586,82.4367265459332,
36.4844843796841));
#167403=CARTESIAN_POINT('Ctrl Pts',(-0.223780545620187,82.4172783657563,
36.448101003167));
#167404=CARTESIAN_POINT('Ctrl Pts',(-0.239161970832704,82.4130622602264,
36.4402246381295));
#167405=CARTESIAN_POINT('Ctrl Pts',(-0.253999999999999,82.4084671089001,
36.4316578979955));
#167406=CARTESIAN_POINT('Ctrl Pts',(-2.778125,81.9939,34.9743536497773));
#167407=CARTESIAN_POINT('Ctrl Pts',(-1.59266295510978,81.9939,35.6587804805087));
#167408=CARTESIAN_POINT('Ctrl Pts',(-0.253999999999474,82.4084671089003,
36.4316578979959));
#167409=CARTESIAN_POINT('Origin',(0.,81.9939,30.1625));
#167410=CARTESIAN_POINT('',(5.55625,82.4084671089001,33.0771084964365));
#167411=CARTESIAN_POINT('Ctrl Pts',(5.55625,82.4084671089003,33.0771084964372));
#167412=CARTESIAN_POINT('Ctrl Pts',(5.55625,81.9939,31.5313536614629));
#167413=CARTESIAN_POINT('Ctrl Pts',(5.55625,81.9939,30.1625));
#167414=CARTESIAN_POINT('',(5.30225000000001,82.4084671089001,33.517049401559));
#167415=CARTESIAN_POINT('Ctrl Pts',(5.55625,82.4084671089001,33.0771084964365));
#167416=CARTESIAN_POINT('Ctrl Pts',(5.55625,82.4130622602264,33.0942419767045));
#167417=CARTESIAN_POINT('Ctrl Pts',(5.55538041960568,82.4172783657563,33.1115008642037));
#167418=CARTESIAN_POINT('Ctrl Pts',(5.54634893312311,82.4367265459332,33.1999106106935));
#167419=CARTESIAN_POINT('Ctrl Pts',(5.52304236276573,82.4447915035635,33.2707440010806));
#167420=CARTESIAN_POINT('Ctrl Pts',(5.45333944747927,82.4447915035635,33.3914729917924));
#167421=CARTESIAN_POINT('Ctrl Pts',(5.40364921714653,82.4367265459332,33.4470737689906));
#167422=CARTESIAN_POINT('Ctrl Pts',(5.3315998739855,82.4172783657563,33.4991001389633));
#167423=CARTESIAN_POINT('Ctrl Pts',(5.3170880291673,82.4130622602264,33.508482661425));
#167424=CARTESIAN_POINT('Ctrl Pts',(5.30225000000001,82.4084671089001,33.517049401559));
#167425=CARTESIAN_POINT('Ctrl Pts',(2.77812500000001,81.9939,34.9743536497773));
#167426=CARTESIAN_POINT('Ctrl Pts',(3.96358704489023,81.9939,34.2899268190458));
#167427=CARTESIAN_POINT('Ctrl Pts',(5.30225000000053,82.4084671089003,33.5170494015587));
#167428=CARTESIAN_POINT('Origin',(0.,81.9939,30.1625));
#167429=CARTESIAN_POINT('',(5.30225000000253,82.4084671089009,26.8079505984424));
#167430=CARTESIAN_POINT('Ctrl Pts',(5.30225000000308,82.4084671089011,26.8079505984428));
#167431=CARTESIAN_POINT('Ctrl Pts',(3.96358704489129,81.9939,26.0350731809548));
#167432=CARTESIAN_POINT('Ctrl Pts',(2.77812500000002,81.9939,25.3506463502227));
#167433=CARTESIAN_POINT('',(5.55625,82.4084671089002,27.2478915035631));
#167434=CARTESIAN_POINT('Ctrl Pts',(5.30225000000254,82.4084671089009,26.8079505984424));
#167435=CARTESIAN_POINT('Ctrl Pts',(5.31708802916896,82.4130622602269,26.816517338576));
#167436=CARTESIAN_POINT('Ctrl Pts',(5.33159987398629,82.4172783657565,26.8258998610373));
#167437=CARTESIAN_POINT('Ctrl Pts',(5.40364921714653,82.4367265459332,26.8779262310094));
#167438=CARTESIAN_POINT('Ctrl Pts',(5.45333944747927,82.4447915035635,26.9335270082076));
#167439=CARTESIAN_POINT('Ctrl Pts',(5.52304236276573,82.4447915035635,27.0542559989194));
#167440=CARTESIAN_POINT('Ctrl Pts',(5.54634893312311,82.4367265459332,27.1250893893065));
#167441=CARTESIAN_POINT('Ctrl Pts',(5.55538041960567,82.4172783657563,27.2134991357962));
#167442=CARTESIAN_POINT('Ctrl Pts',(5.55624999999999,82.4130622602265,27.2307580232952));
#167443=CARTESIAN_POINT('Ctrl Pts',(5.55625,82.4084671089002,27.2478915035631));
#167444=CARTESIAN_POINT('Ctrl Pts',(5.55625,81.9939,30.1625));
#167445=CARTESIAN_POINT('Ctrl Pts',(5.55625,81.9939,28.7936463385369));
#167446=CARTESIAN_POINT('Ctrl Pts',(5.55625,82.4084671089004,27.2478915035625));
#167447=CARTESIAN_POINT('Origin',(0.,85.9309,23.7466951336303));
#167448=CARTESIAN_POINT('',(5.30225,85.9309,26.807950598441));
#167449=CARTESIAN_POINT('Origin',(5.55625,85.9309,26.9545975668151));
#167450=CARTESIAN_POINT('',(5.55625,85.9309,27.2478915035635));
#167451=CARTESIAN_POINT('',(5.55625,85.9309,33.0771084964365));
#167452=CARTESIAN_POINT('Origin',(0.,85.9309,36.5783048663697));
#167453=CARTESIAN_POINT('',(5.30225,85.9309,33.517049401559));
#167454=CARTESIAN_POINT('',(0.254000000000001,85.9309,36.4316578979955));
#167455=CARTESIAN_POINT('Origin',(-5.55625,85.9309,33.3704024331849));
#167456=CARTESIAN_POINT('',(-5.30225,85.9309,33.517049401559));
#167457=CARTESIAN_POINT('',(-0.254000000000001,85.9309,36.4316578979955));
#167458=CARTESIAN_POINT('Origin',(-5.55625,85.9309,26.9545975668151));
#167459=CARTESIAN_POINT('',(-5.55625,85.9309,27.2478915035635));
#167460=CARTESIAN_POINT('',(-5.55625,85.9309,33.0771084964365));
#167461=CARTESIAN_POINT('Origin',(-5.55625,85.9309,26.9545975668151));
#167462=CARTESIAN_POINT('',(-5.30225,85.9309,26.807950598441));
#167463=CARTESIAN_POINT('Origin',(5.04825,85.9309,27.2478915035635));
#167464=CARTESIAN_POINT('Origin',(-5.04825,85.9309,27.2478915035635));
#167465=CARTESIAN_POINT('Origin',(-5.04825,85.9309,33.0771084964365));
#167466=CARTESIAN_POINT('Origin',(5.04825,85.9309,33.0771084964365));
#167467=CARTESIAN_POINT('Origin',(-6.50521303491303E-16,85.9309,35.9917169928731));
#167468=CARTESIAN_POINT('Origin',(90.,90.,41.3499812820439));
#167469=CARTESIAN_POINT('',(97.9375,90.,17.4625));
#167470=CARTESIAN_POINT('Origin',(90.,90.,17.4625));
#167471=CARTESIAN_POINT('',(97.9375,90.,3.17499999999999));
#167472=CARTESIAN_POINT('',(97.9375,90.,41.3499812820439));
#167473=CARTESIAN_POINT('Origin',(90.,90.,3.175));
#167474=CARTESIAN_POINT('Origin',(90.,90.,41.3499812820439));
#167475=CARTESIAN_POINT('',(98.4455,90.,3.175));
#167476=CARTESIAN_POINT('Origin',(90.,90.,3.175));
#167477=CARTESIAN_POINT('',(98.4455,90.,17.4625));
#167478=CARTESIAN_POINT('',(98.4455,90.,41.3499812820439));
#167479=CARTESIAN_POINT('Origin',(90.,90.,17.4625));
#167480=CARTESIAN_POINT('Origin',(90.,90.,3.175));
#167481=CARTESIAN_POINT('Origin',(-90.,-90.,17.4625));
#167482=CARTESIAN_POINT('Origin',(-90.,90.,41.3499812820439));
#167483=CARTESIAN_POINT('',(-82.0625,90.,17.4625));
#167484=CARTESIAN_POINT('Origin',(-90.,90.,17.4625));
#167485=CARTESIAN_POINT('',(-82.0625,90.,3.17499999999999));
#167486=CARTESIAN_POINT('',(-82.0625,90.,41.3499812820439));
#167487=CARTESIAN_POINT('Origin',(-90.,90.,3.175));
#167488=CARTESIAN_POINT('Origin',(-90.,90.,41.3499812820439));
#167489=CARTESIAN_POINT('',(-81.5545,90.,3.175));
#167490=CARTESIAN_POINT('Origin',(-90.,90.,3.175));
#167491=CARTESIAN_POINT('',(-81.5545,90.,17.4625));
#167492=CARTESIAN_POINT('',(-81.5545,90.,41.3499812820439));
#167493=CARTESIAN_POINT('Origin',(-90.,90.,17.4625));
#167494=CARTESIAN_POINT('Origin',(-90.,90.,3.175));
#167495=CARTESIAN_POINT('Origin',(-90.,-90.,17.4625));
#167496=CARTESIAN_POINT('Origin',(-90.,-90.,41.3499812820439));
#167497=CARTESIAN_POINT('',(-82.0625,-90.,17.4625));
#167498=CARTESIAN_POINT('Origin',(-90.,-90.,17.4625));
#167499=CARTESIAN_POINT('',(-82.0625,-90.,3.17499999999999));
#167500=CARTESIAN_POINT('',(-82.0625,-90.,41.3499812820439));
#167501=CARTESIAN_POINT('Origin',(-90.,-90.,3.175));
#167502=CARTESIAN_POINT('Origin',(-90.,-90.,41.3499812820439));
#167503=CARTESIAN_POINT('',(-81.5545,-90.,3.175));
#167504=CARTESIAN_POINT('Origin',(-90.,-90.,3.175));
#167505=CARTESIAN_POINT('',(-81.5545,-90.,17.4625));
#167506=CARTESIAN_POINT('',(-81.5545,-90.,41.3499812820439));
#167507=CARTESIAN_POINT('Origin',(-90.,-90.,17.4625));
#167508=CARTESIAN_POINT('Origin',(-90.,-90.,3.175));
#167509=CARTESIAN_POINT('Origin',(-90.,-90.,17.4625));
#167510=CARTESIAN_POINT('Origin',(90.,-90.,41.3499812820439));
#167511=CARTESIAN_POINT('',(97.9375,-90.,17.4625));
#167512=CARTESIAN_POINT('Origin',(90.,-90.,17.4625));
#167513=CARTESIAN_POINT('',(97.9375,-90.,3.17499999999999));
#167514=CARTESIAN_POINT('',(97.9375,-90.,41.3499812820439));
#167515=CARTESIAN_POINT('Origin',(90.,-90.,3.175));
#167516=CARTESIAN_POINT('Origin',(90.,-90.,41.3499812820439));
#167517=CARTESIAN_POINT('',(98.4455,-90.,3.175));
#167518=CARTESIAN_POINT('Origin',(90.,-90.,3.175));
#167519=CARTESIAN_POINT('',(98.4455,-90.,17.4625));
#167520=CARTESIAN_POINT('',(98.4455,-90.,41.3499812820439));
#167521=CARTESIAN_POINT('Origin',(90.,-90.,17.4625));
#167522=CARTESIAN_POINT('Origin',(90.,-90.,3.175));
#167523=CARTESIAN_POINT('Origin',(-90.,-90.,17.4625));
#167524=CARTESIAN_POINT('Origin',(-1.38777878078145E-14,-1.38777878078145E-14,
2.79399999999999));
#167525=CARTESIAN_POINT('',(-50.,-7.75455381207769E-15,2.79399999999999));
#167526=CARTESIAN_POINT('',(50.,-2.00010218035512E-14,2.79399999999999));
#167527=CARTESIAN_POINT('Origin',(-1.38777878078145E-14,-1.38777878078145E-14,
2.79399999999999));
#167528=CARTESIAN_POINT('Origin',(-1.38777878078145E-14,-1.38777878078145E-14,
2.79399999999999));
#167529=CARTESIAN_POINT('',(50.254,-2.00321278322496E-14,2.54));
#167530=CARTESIAN_POINT('Origin',(50.254,-2.00321278322496E-14,2.79399999999999));
#167531=CARTESIAN_POINT('Origin',(-1.38777878078145E-14,-1.38777878078145E-14,
2.54));
#167532=CARTESIAN_POINT('Origin',(-1.38777878078145E-14,-1.38777878078145E-14,
2.79399999999999));
#167533=CARTESIAN_POINT('',(51.016,-2.01254459183446E-14,2.54));
#167534=CARTESIAN_POINT('Origin',(-1.38777878078145E-14,-1.38777878078145E-14,
2.54));
#167535=CARTESIAN_POINT('',(51.27,-2.01565519470429E-14,2.79399999999999));
#167536=CARTESIAN_POINT('Origin',(51.016,-2.01254459183446E-14,2.79399999999999));
#167537=CARTESIAN_POINT('',(-51.27,-7.59902366858598E-15,2.79399999999999));
#167538=CARTESIAN_POINT('Origin',(-1.38777878078145E-14,-1.38777878078145E-14,
2.79399999999999));
#167539=CARTESIAN_POINT('Origin',(-1.38777878078145E-14,-1.38777878078145E-14,
2.79399999999999));
#167540=CARTESIAN_POINT('Origin',(-1.38777878078145E-14,-1.38777878078145E-14,
-158.32679271994));
#167541=CARTESIAN_POINT('',(-51.27,-2.01565519470429E-14,17.4625));
#167542=CARTESIAN_POINT('Origin',(-1.38777878078145E-14,-1.38777878078145E-14,
17.4625));
#167543=CARTESIAN_POINT('',(-51.27,-2.01565519470429E-14,-158.32679271994));
#167544=CARTESIAN_POINT('Origin',(-1.38777878078145E-14,-1.38777878078145E-14,
-158.32679271994));
#167545=CARTESIAN_POINT('',(-50.,-2.00010218035512E-14,17.4625));
#167546=CARTESIAN_POINT('',(-50.,-2.00010218035512E-14,-158.32679271994));
#167547=CARTESIAN_POINT('Origin',(-1.38777878078145E-14,-1.38777878078145E-14,
17.4625));
#167548=CARTESIAN_POINT('Origin',(0.,0.,17.4625));
#167549=CARTESIAN_POINT('Origin',(-90.,-90.,2.54));
#167550=CARTESIAN_POINT('Origin',(-1.38777878078145E-14,-1.38777878078145E-14,
2.79399999999999));
#167551=CARTESIAN_POINT('',(56.621,-2.08118604492667E-14,2.54));
#167552=CARTESIAN_POINT('Origin',(-1.38777878078145E-14,-1.38777878078145E-14,
2.54));
#167553=CARTESIAN_POINT('',(56.875,-2.0842966477965E-14,2.79399999999999));
#167554=CARTESIAN_POINT('Origin',(56.621,-2.08118604492667E-14,2.79399999999999));
#167555=CARTESIAN_POINT('',(-56.875,-6.91260913766388E-15,2.79399999999999));
#167556=CARTESIAN_POINT('Origin',(-1.38777878078145E-14,-1.38777878078145E-14,
2.79399999999999));
#167557=CARTESIAN_POINT('Origin',(-1.38777878078145E-14,-1.38777878078145E-14,
2.79399999999999));
#167558=CARTESIAN_POINT('Origin',(-1.38777878078145E-14,-1.38777878078145E-14,
2.79399999999999));
#167559=CARTESIAN_POINT('',(-55.605,-7.0681392811556E-15,2.79399999999999));
#167560=CARTESIAN_POINT('',(55.605,-2.06874363344733E-14,2.79399999999999));
#167561=CARTESIAN_POINT('Origin',(-1.38777878078145E-14,-1.38777878078145E-14,
2.79399999999999));
#167562=CARTESIAN_POINT('Origin',(-1.38777878078145E-14,-1.38777878078145E-14,
2.79399999999999));
#167563=CARTESIAN_POINT('',(55.859,-2.07185423631717E-14,2.54));
#167564=CARTESIAN_POINT('Origin',(55.859,-2.07185423631717E-14,2.79399999999999));
#167565=CARTESIAN_POINT('Origin',(-1.38777878078145E-14,-1.38777878078145E-14,
2.54));
#167566=CARTESIAN_POINT('Origin',(-1.38777878078145E-14,-1.38777878078145E-14,
-158.32679271994));
#167567=CARTESIAN_POINT('',(-56.875,-2.0842966477965E-14,17.4625));
#167568=CARTESIAN_POINT('Origin',(-1.38777878078145E-14,-1.38777878078145E-14,
17.4625));
#167569=CARTESIAN_POINT('',(-56.875,-2.0842966477965E-14,-158.32679271994));
#167570=CARTESIAN_POINT('Origin',(-1.38777878078145E-14,-1.38777878078145E-14,
-158.32679271994));
#167571=CARTESIAN_POINT('',(-55.605,-2.06874363344733E-14,17.4625));
#167572=CARTESIAN_POINT('',(-55.605,-2.06874363344733E-14,-158.32679271994));
#167573=CARTESIAN_POINT('Origin',(-1.38777878078145E-14,-1.38777878078145E-14,
17.4625));
#167574=CARTESIAN_POINT('Origin',(0.,0.,17.4625));
#167575=CARTESIAN_POINT('Origin',(-90.,-90.,2.54));
#167576=CARTESIAN_POINT('Origin',(-1.38777878078145E-14,-1.38777878078145E-14,
-154.734690271512));
#167577=CARTESIAN_POINT('',(-51.27,-2.01565519470429E-14,2.53999999999998));
#167578=CARTESIAN_POINT('Origin',(-1.38777878078145E-14,-1.38777878078145E-14,
2.53999999999999));
#167579=CARTESIAN_POINT('',(-51.27,-2.01565519470429E-14,17.4625));
#167580=CARTESIAN_POINT('',(-51.27,-2.01565519470429E-14,-154.734690271512));
#167581=CARTESIAN_POINT('Origin',(-1.38777878078145E-14,-1.38777878078145E-14,
17.4625));
#167582=CARTESIAN_POINT('Origin',(-1.38777878078145E-14,-1.38777878078145E-14,
-154.734690271512));
#167583=CARTESIAN_POINT('',(-55.605,-2.06874363344733E-14,17.4625));
#167584=CARTESIAN_POINT('Origin',(-1.38777878078145E-14,-1.38777878078145E-14,
17.4625));
#167585=CARTESIAN_POINT('',(-55.605,-2.06874363344733E-14,2.53999999999998));
#167586=CARTESIAN_POINT('',(-55.605,-2.06874363344733E-14,-154.734690271512));
#167587=CARTESIAN_POINT('Origin',(-1.38777878078145E-14,-1.38777878078145E-14,
2.53999999999999));
#167588=CARTESIAN_POINT('Origin',(-1.38777878078145E-14,-1.38777878078145E-14,
17.4625));
#167589=CARTESIAN_POINT('Origin',(-90.,-90.,2.54));
#167590=CARTESIAN_POINT('Origin',(5.66467691768715E-15,5.31136514129714E-15,
40.22725));
#167591=CARTESIAN_POINT('',(-0.0152399999993761,59.0285534841296,40.10025));
#167592=CARTESIAN_POINT('',(0.0152400000006239,59.0285534841296,40.10025));
#167593=CARTESIAN_POINT('Origin',(5.64679317051214E-15,5.32924888847216E-15,
40.10025));
#167594=CARTESIAN_POINT('',(-0.015212193455297,58.9208513795073,40.1599502534424));
#167595=CARTESIAN_POINT('Origin',(-0.015239999999376,59.0285534841296,40.22725));
#167596=CARTESIAN_POINT('',(0.0152121934565426,58.9208513795073,40.1599502534424));
#167597=CARTESIAN_POINT('Origin',(5.65519997554244E-15,5.32084208344186E-15,
40.1599502534424));
#167598=CARTESIAN_POINT('Origin',(0.0152400000006239,59.0285534841296,40.22725));
#167599=CARTESIAN_POINT('Origin',(5.66467691768715E-15,5.52999499151977E-15,
40.22725));
#167600=CARTESIAN_POINT('',(-0.0152661173102018,62.9541448057648,40.1599502534424));
#167601=CARTESIAN_POINT('',(0.0152661173115319,62.9541448057648,40.1599502534424));
#167602=CARTESIAN_POINT('Origin',(5.65519997554243E-15,5.53947193366449E-15,
40.1599502534424));
#167603=CARTESIAN_POINT('',(-0.0152399999993361,62.8464427007196,40.10025));
#167604=CARTESIAN_POINT('Origin',(-0.015239999999336,62.8464427007196,40.22725));
#167605=CARTESIAN_POINT('',(0.0152400000006639,62.8464427007196,40.10025));
#167606=CARTESIAN_POINT('Origin',(5.64679317051213E-15,5.54787873869479E-15,
40.10025));
#167607=CARTESIAN_POINT('Origin',(0.0152400000006639,62.8464427007196,40.22725));
#167608=CARTESIAN_POINT('Origin',(3.5331177639001E-16,0.,40.22725));
#167609=CARTESIAN_POINT('',(-59.0285534841296,-0.01524,40.10025));
#167610=CARTESIAN_POINT('',(-59.0285534841296,0.01524,40.10025));
#167611=CARTESIAN_POINT('Origin',(3.17544282039971E-16,0.,40.10025));
#167612=CARTESIAN_POINT('',(-58.9208513795073,-0.0152121934559198,40.1599502534424));
#167613=CARTESIAN_POINT('Origin',(-59.0285534841296,-0.01524,40.22725));
#167614=CARTESIAN_POINT('',(-58.9208513795073,0.0152121934559198,40.1599502534424));
#167615=CARTESIAN_POINT('Origin',(3.34357892100574E-16,0.,40.1599502534424));
#167616=CARTESIAN_POINT('Origin',(-59.0285534841296,0.01524,40.22725));
#167617=CARTESIAN_POINT('Origin',(1.34681926167381E-16,0.,40.22725));
#167618=CARTESIAN_POINT('',(-62.9541448057648,-0.0152661173108668,40.1599502534424));
#167619=CARTESIAN_POINT('',(-62.9541466567496,-7.70965941962415E-15,40.1599502534424));
#167620=CARTESIAN_POINT('Origin',(1.15728041877948E-16,0.,40.1599502534424));
#167621=CARTESIAN_POINT('',(-62.8464427007196,-0.01524,40.10025));
#167622=CARTESIAN_POINT('Origin',(-62.8464427007196,-0.01524,40.22725));
#167623=CARTESIAN_POINT('',(-62.8464427007196,0.01524,40.10025));
#167624=CARTESIAN_POINT('Origin',(9.89144318173425E-17,0.,40.10025));
#167625=CARTESIAN_POINT('',(-62.9541448057648,0.0152661173108668,40.1599502534424));
#167626=CARTESIAN_POINT('Origin',(-62.8464427007196,0.01524,40.22725));
#167627=CARTESIAN_POINT('Origin',(1.15728041877948E-16,0.,40.1599502534424));
#167628=CARTESIAN_POINT('Origin',(5.62443848654336E-15,0.,39.9415));
#167629=CARTESIAN_POINT('',(58.2189663438286,-7.12976707826372E-15,40.5765));
#167630=CARTESIAN_POINT('Origin',(5.71385722241845E-15,0.,40.5765));
#167631=CARTESIAN_POINT('',(57.6804558027693,-7.06381855722217E-15,40.2779987327881));
#167632=CARTESIAN_POINT('Origin',(58.2189663438286,-7.12976707826372E-15,
39.9415));
#167633=CARTESIAN_POINT('',(-57.6804558027693,7.06381855722218E-15,40.2779987327881));
#167634=CARTESIAN_POINT('Origin',(5.67182319726696E-15,0.,40.2779987327881));
#167635=CARTESIAN_POINT('Origin',(5.67182319726696E-15,0.,40.2779987327881));
#167636=CARTESIAN_POINT('Origin',(5.62443848654336E-15,0.,39.9415));
#167637=CARTESIAN_POINT('',(58.8470884664677,-7.20668985296008E-15,40.2779987327881));
#167638=CARTESIAN_POINT('Origin',(5.67182319726695E-15,0.,40.2779987327881));
#167639=CARTESIAN_POINT('',(58.3085779254084,-7.14074133191854E-15,40.5765));
#167640=CARTESIAN_POINT('Origin',(58.3085779254084,-7.14074133191854E-15,
39.9415));
#167641=CARTESIAN_POINT('Origin',(5.71385722241845E-15,0.,40.5765));
#167642=CARTESIAN_POINT('Origin',(5.62443848654336E-15,0.,39.9415));
#167643=CARTESIAN_POINT('',(63.5664220745916,-7.78464153268983E-15,40.5765));
#167644=CARTESIAN_POINT('Origin',(5.71385722241845E-15,0.,40.5765));
#167645=CARTESIAN_POINT('',(63.0279115335323,-7.71869301164828E-15,40.2779987327881));
#167646=CARTESIAN_POINT('Origin',(63.5664220745916,-7.78464153268983E-15,
39.9415));
#167647=CARTESIAN_POINT('',(-63.0279115335323,7.71869301164829E-15,40.2779987327881));
#167648=CARTESIAN_POINT('Origin',(5.67182319726696E-15,0.,40.2779987327881));
#167649=CARTESIAN_POINT('Origin',(5.67182319726696E-15,0.,40.2779987327881));
#167650=CARTESIAN_POINT('Origin',(5.62443848654336E-15,0.,39.9415));
#167651=CARTESIAN_POINT('',(64.1945441972308,-7.8615643073862E-15,40.2779987327881));
#167652=CARTESIAN_POINT('Origin',(5.67182319726695E-15,0.,40.2779987327881));
#167653=CARTESIAN_POINT('',(63.6560336561714,-7.79561578634465E-15,40.5765));
#167654=CARTESIAN_POINT('Origin',(63.6560336561714,-7.79561578634465E-15,
39.9415));
#167655=CARTESIAN_POINT('Origin',(5.71385722241845E-15,0.,40.5765));
#167656=CARTESIAN_POINT('Origin',(0.,0.,0.));
#167657=CARTESIAN_POINT('',(65.,-7.96020419445779E-15,38.6715));
#167658=CARTESIAN_POINT('Origin',(5.44560101479317E-15,0.,38.6715));
#167659=CARTESIAN_POINT('',(65.,-7.96020419445779E-15,38.989));
#167660=CARTESIAN_POINT('',(65.,-7.96020419445779E-15,-9.15309894784418E-15));
#167661=CARTESIAN_POINT('Origin',(5.49031038273072E-15,0.,38.989));
#167662=CARTESIAN_POINT('Origin',(5.71385722241845E-15,0.,40.5765));
#167663=CARTESIAN_POINT('',(64.008019903844,-7.83872166950026E-15,40.5765));
#167664=CARTESIAN_POINT('Origin',(5.49031038273072E-15,0.,38.989));
#167665=CARTESIAN_POINT('',(62.9541448057648,0.0152661173108668,40.1599502534424));
#167666=CARTESIAN_POINT('',(62.9541448057648,-0.0152661173108668,40.1599502534424));
#167667=CARTESIAN_POINT('Origin',(-1.95097259456047E-16,0.,40.1599502534424));
#167668=CARTESIAN_POINT('',(62.7644678366119,-0.318045750793045,39.8576902534424));
#167669=CARTESIAN_POINT('Ctrl Pts',(62.9541448057648,-0.0152661173108668,
40.1599502534424));
#167670=CARTESIAN_POINT('Ctrl Pts',(62.9541438736292,-0.019087735244646,
40.1599502447858));
#167671=CARTESIAN_POINT('Ctrl Pts',(62.9540952129414,-0.0228988721022198,
40.1598744685927));
#167672=CARTESIAN_POINT('Ctrl Pts',(62.9539999459718,-0.0266975986403399,
40.1597246934279));
#167673=CARTESIAN_POINT('Ctrl Pts',(62.953449420412,-0.0486495517930185,
40.1588591777434));
#167674=CARTESIAN_POINT('Ctrl Pts',(62.9513443281453,-0.0701898812469889,
40.1555254706015));
#167675=CARTESIAN_POINT('Ctrl Pts',(62.9479003565106,-0.0909392844447056,
40.1500631826367));
#167676=CARTESIAN_POINT('Ctrl Pts',(62.9465113235258,-0.0993079960697583,
40.1478601162471));
#167677=CARTESIAN_POINT('Ctrl Pts',(62.9449047668209,-0.107548428339421,
40.1453112228301));
#167678=CARTESIAN_POINT('Ctrl Pts',(62.9430957254317,-0.115637319282189,
40.1424401896328));
#167679=CARTESIAN_POINT('Ctrl Pts',(62.9424282989905,-0.118621628943446,
40.1413809526906));
#167680=CARTESIAN_POINT('Ctrl Pts',(62.9417332466658,-0.121585194085533,
40.1402777640512));
#167681=CARTESIAN_POINT('Ctrl Pts',(62.941011293136,-0.124526788072755,
40.1391317641987));
#167682=CARTESIAN_POINT('Ctrl Pts',(62.9396576302675,-0.130042276798797,
40.1369830144753));
#167683=CARTESIAN_POINT('Ctrl Pts',(62.938209392844,-0.135480523183572,
40.134683756585));
#167684=CARTESIAN_POINT('Ctrl Pts',(62.9366713579026,-0.14083344149334,
40.1322415082996));
#167685=CARTESIAN_POINT('Ctrl Pts',(62.9312882356078,-0.159568655577527,
40.1236936393009));
#167686=CARTESIAN_POINT('Ctrl Pts',(62.9248050892389,-0.177258600738952,
40.113394140767));
#167687=CARTESIAN_POINT('Ctrl Pts',(62.9174267595942,-0.193556601113636,
40.101665321223));
#167688=CARTESIAN_POINT('Ctrl Pts',(62.9137375947718,-0.201705601300978,
40.095800911451));
#167689=CARTESIAN_POINT('Ctrl Pts',(62.9098246351408,-0.209506615291396,
40.0895791707949));
#167690=CARTESIAN_POINT('Ctrl Pts',(62.9057134946881,-0.216916308650389,
40.0830403822906));
#167691=CARTESIAN_POINT('Ctrl Pts',(62.9036579244618,-0.220621155329885,
40.0797709880385));
#167692=CARTESIAN_POINT('Ctrl Pts',(62.9015528091474,-0.224228171852543,
40.0764223317514));
#167693=CARTESIAN_POINT('Ctrl Pts',(62.8994013510256,-0.227731941419532,
40.0729994484778));
#167694=CARTESIAN_POINT('Ctrl Pts',(62.8972498929038,-0.231235710986522,
40.0695765652042));
#167695=CARTESIAN_POINT('Ctrl Pts',(62.8950520414621,-0.234636114276735,
40.0660793733488));
#167696=CARTESIAN_POINT('Ctrl Pts',(62.8928111037451,-0.237927978230923,
40.0625130768817));
#167697=CARTESIAN_POINT('Ctrl Pts',(62.8927919932396,-0.237956050936217,
40.0624826638418));
#167698=CARTESIAN_POINT('Ctrl Pts',(62.8927728797351,-0.237984115711008,
40.0624522459912));
#167699=CARTESIAN_POINT('Ctrl Pts',(62.8927537632335,-0.238012172552841,
40.0624218233329));
#167700=CARTESIAN_POINT('Ctrl Pts',(62.882990686785,-0.252341211296126,
40.0468845275922));
#167701=CARTESIAN_POINT('Ctrl Pts',(62.8725309380423,-0.264702219189255,
40.0302263329287));
#167702=CARTESIAN_POINT('Ctrl Pts',(62.8615664772849,-0.275152816745115,
40.0127515884821));
#167703=CARTESIAN_POINT('Ctrl Pts',(62.8502312057454,-0.285956846570894,
39.994685859782));
#167704=CARTESIAN_POINT('Ctrl Pts',(62.8383556508917,-0.294719332055952,
39.9757460620624));
#167705=CARTESIAN_POINT('Ctrl Pts',(62.8261370346475,-0.301453885678947,
39.9562444559293));
#167706=CARTESIAN_POINT('Ctrl Pts',(62.8141508421947,-0.308060333921169,
39.9371138113801));
#167707=CARTESIAN_POINT('Ctrl Pts',(62.8018335935216,-0.312715155744622,
39.9174410654569));
#167708=CARTESIAN_POINT('Ctrl Pts',(62.7893708783698,-0.315383336840266,
39.8975196504386));
#167709=CARTESIAN_POINT('Ctrl Pts',(62.7811147664994,-0.31715091327508,
39.8843224113936));
#167710=CARTESIAN_POINT('Ctrl Pts',(62.7727948225175,-0.318045664008453,
39.8710160447212));
#167711=CARTESIAN_POINT('Ctrl Pts',(62.7644678366119,-0.318045750793045,
39.8576902534424));
#167712=CARTESIAN_POINT('',(62.4081695979768,-0.318048871877129,39.2875012672119));
#167713=CARTESIAN_POINT('',(62.7644678366119,-0.318045750793045,39.8576902534424));
#167714=CARTESIAN_POINT('',(62.0995362748659,-6.20712349654464,39.2875012672119));
#167715=CARTESIAN_POINT('Origin',(5.53234440788222E-15,0.,39.2875012672119));
#167716=CARTESIAN_POINT('',(62.4538823482275,-6.2443699078806,39.8576902534424));
#167717=CARTESIAN_POINT('',(62.0995362748659,-6.20712349654464,39.2875012672119));
#167718=CARTESIAN_POINT('',(62.6108711573006,-6.56531752495302,40.1599502534424));
#167719=CARTESIAN_POINT('Ctrl Pts',(62.4538823482275,-6.2443699078806,39.8576902534424));
#167720=CARTESIAN_POINT('Ctrl Pts',(62.4661208561102,-6.2456563596144,39.8773836120348));
#167721=CARTESIAN_POINT('Ctrl Pts',(62.4781153572947,-6.24887816048055,
39.8969946442101));
#167722=CARTESIAN_POINT('Ctrl Pts',(62.489703469055,-6.25393874389324,39.9162525288194));
#167723=CARTESIAN_POINT('Ctrl Pts',(62.5015244311524,-6.25910101415343,
39.9358973794));
#167724=CARTESIAN_POINT('Ctrl Pts',(62.5129234356945,-6.26617675898116,
39.9551762199662));
#167725=CARTESIAN_POINT('Ctrl Pts',(62.523731436973,-6.27511683300192,39.9738152034151));
#167726=CARTESIAN_POINT('Ctrl Pts',(62.5341195571996,-6.28370959325135,
39.9917300792536));
#167727=CARTESIAN_POINT('Ctrl Pts',(62.5439624606626,-6.29402509233189,
40.0090551157999));
#167728=CARTESIAN_POINT('Ctrl Pts',(62.5531007542688,-6.30606398946847,
40.02553945514));
#167729=CARTESIAN_POINT('Ctrl Pts',(62.5601204743137,-6.31531185249311,
40.0382021526063));
#167730=CARTESIAN_POINT('Ctrl Pts',(62.5667243349245,-6.32557753707731,
40.0503687782082));
#167731=CARTESIAN_POINT('Ctrl Pts',(62.5728320301413,-6.33687803771691,
40.0619155352442));
#167732=CARTESIAN_POINT('Ctrl Pts',(62.5728480373212,-6.33690765431375,
40.0619457972351));
#167733=CARTESIAN_POINT('Ctrl Pts',(62.5728640408535,-6.33693727882097,
40.0619760547304));
#167734=CARTESIAN_POINT('Ctrl Pts',(62.5728800407364,-6.33696691123577,
40.0620063077269));
#167735=CARTESIAN_POINT('Ctrl Pts',(62.5745955535553,-6.34014410870328,
40.06525004417));
#167736=CARTESIAN_POINT('Ctrl Pts',(62.5762674929177,-6.34341121944319,
40.0684393223556));
#167737=CARTESIAN_POINT('Ctrl Pts',(62.5778935423008,-6.34676388583387,
40.0715697951759));
#167738=CARTESIAN_POINT('Ctrl Pts',(62.586942137402,-6.36542071200092,40.0889901646436));
#167739=CARTESIAN_POINT('Ctrl Pts',(62.5945741278866,-6.38672471011642,
40.104596309827));
#167740=CARTESIAN_POINT('Ctrl Pts',(62.600410948358,-6.40987366744635,40.117663465076));
#167741=CARTESIAN_POINT('Ctrl Pts',(62.603030594215,-6.42026324006751,40.1235281853083));
#167742=CARTESIAN_POINT('Ctrl Pts',(62.6052889671231,-6.43102458681719,
40.1288820140929));
#167743=CARTESIAN_POINT('Ctrl Pts',(62.6071534261453,-6.44208677567865,
40.1336621774101));
#167744=CARTESIAN_POINT('Ctrl Pts',(62.6079636948179,-6.44689425333218,
40.1357395717319));
#167745=CARTESIAN_POINT('Ctrl Pts',(62.6086994224563,-6.45175840517988,
40.1377083672883));
#167746=CARTESIAN_POINT('Ctrl Pts',(62.6093578414453,-6.45667331290429,
40.1395632548791));
#167747=CARTESIAN_POINT('Ctrl Pts',(62.6116623079068,-6.47387548993976,
40.1460553614469));
#167748=CARTESIAN_POINT('Ctrl Pts',(62.6130197402063,-6.49169942613405,
40.1511520974629));
#167749=CARTESIAN_POINT('Ctrl Pts',(62.6133114945132,-6.50989137546619,
40.1546258197408));
#167750=CARTESIAN_POINT('Ctrl Pts',(62.6134573716666,-6.51898735013226,
40.1563626808798));
#167751=CARTESIAN_POINT('Ctrl Pts',(62.6133368299269,-6.52817532814393,
40.1576937882008));
#167752=CARTESIAN_POINT('Ctrl Pts',(62.6129350466932,-6.53742359207002,
40.1585906813668));
#167753=CARTESIAN_POINT('Ctrl Pts',(62.6127341550764,-6.54204772403306,
40.1590391279498));
#167754=CARTESIAN_POINT('Ctrl Pts',(62.6124629532086,-6.54668692748761,
40.1593790209175));
#167755=CARTESIAN_POINT('Ctrl Pts',(62.6121195889602,-6.55133723782952,
40.1596068022931));
#167756=CARTESIAN_POINT('Ctrl Pts',(62.6117762247118,-6.55598754817143,
40.1598345836687));
#167757=CARTESIAN_POINT('Ctrl Pts',(62.6113606963859,-6.56064896522272,
40.1599502506864));
#167758=CARTESIAN_POINT('Ctrl Pts',(62.6108711573006,-6.56531752495302,
40.1599502534424));
#167759=CARTESIAN_POINT('',(62.6076796697354,-6.59568250079886,40.1599502534424));
#167760=CARTESIAN_POINT('Origin',(5.50063869163689E-15,5.71112962987806E-15,
40.1599502534424));
#167761=CARTESIAN_POINT('',(62.3873926810691,-6.87697683366565,39.8576902534424));
#167762=CARTESIAN_POINT('Ctrl Pts',(62.6076796697354,-6.59568250079886,
40.1599502534424));
#167763=CARTESIAN_POINT('Ctrl Pts',(62.6072792748563,-6.59948308607503,
40.1599502447857));
#167764=CARTESIAN_POINT('Ctrl Pts',(62.6068325084578,-6.60326825869922,
40.1598744685927));
#167765=CARTESIAN_POINT('Ctrl Pts',(62.6063406883232,-6.60703621730596,
40.1597246934279));
#167766=CARTESIAN_POINT('Ctrl Pts',(62.6034985746717,-6.62881036976826,
40.1588591777435));
#167767=CARTESIAN_POINT('Ctrl Pts',(62.5991534367855,-6.65001265698081,
40.1555254706025));
#167768=CARTESIAN_POINT('Ctrl Pts',(62.593559428359,-6.67028839971139,40.1500631826393));
#167769=CARTESIAN_POINT('Ctrl Pts',(62.5913032360759,-6.67846607317848,
40.147860116249));
#167770=CARTESIAN_POINT('Ctrl Pts',(62.5888441205341,-6.68649343259762,
40.1453112228312));
#167771=CARTESIAN_POINT('Ctrl Pts',(62.5861994699221,-6.69434891543609,
40.1424401896328));
#167772=CARTESIAN_POINT('Ctrl Pts',(62.5852237544099,-6.69724711167652,
40.1413809526905));
#167773=CARTESIAN_POINT('Ctrl Pts',(62.5842227327444,-6.70012178934728,
40.1402777640511));
#167774=CARTESIAN_POINT('Ctrl Pts',(62.5831972538526,-6.70297180428183,
40.1391317641987));
#167775=CARTESIAN_POINT('Ctrl Pts',(62.5812744809303,-6.70831558228412,
40.1369830144753));
#167776=CARTESIAN_POINT('Ctrl Pts',(62.5792657255654,-6.71357265535385,
40.1346837565849));
#167777=CARTESIAN_POINT('Ctrl Pts',(62.5771765838154,-6.71873548138815,
40.1322415082996));
#167778=CARTESIAN_POINT('Ctrl Pts',(62.5698645876906,-6.73680537250822,
40.1236936393008));
#167779=CARTESIAN_POINT('Ctrl Pts',(62.5615678538928,-6.75372073697203,
40.113394140767));
#167780=CARTESIAN_POINT('Ctrl Pts',(62.5525263385764,-6.76915820973612,
40.101665321223));
#167781=CARTESIAN_POINT('Ctrl Pts',(62.5480055809182,-6.77687694611817,
40.095800911451));
#167782=CARTESIAN_POINT('Ctrl Pts',(62.5432986288851,-6.78422620968065,
40.0895791707949));
#167783=CARTESIAN_POINT('Ctrl Pts',(62.5384354858299,-6.79116558077034,
40.0830403822906));
#167784=CARTESIAN_POINT('Ctrl Pts',(62.5360039143023,-6.79463526631518,
40.0797709880385));
#167785=CARTESIAN_POINT('Ctrl Pts',(62.5335332951358,-6.7980024787551,40.0764223317514));
#167786=CARTESIAN_POINT('Ctrl Pts',(62.5310273792782,-6.80126216569454,
40.0729994484778));
#167787=CARTESIAN_POINT('Ctrl Pts',(62.5285214634206,-6.80452185263398,
40.0695765652042));
#167788=CARTESIAN_POINT('Ctrl Pts',(62.5259802131086,-6.80767389012548,
40.0660793733488));
#167789=CARTESIAN_POINT('Ctrl Pts',(62.5234074580025,-6.81071347912866,
40.0625130768816));
#167790=CARTESIAN_POINT('Ctrl Pts',(62.5233855177896,-6.81073940045697,
40.0624826638418));
#167791=CARTESIAN_POINT('Ctrl Pts',(62.5233635754231,-6.81076531358473,
40.0624522459912));
#167792=CARTESIAN_POINT('Ctrl Pts',(62.5233416309052,-6.81079121850972,
40.0624218233329));
#167793=CARTESIAN_POINT('Ctrl Pts',(62.5121342452084,-6.82402124190459,
40.0468845275886));
#167794=CARTESIAN_POINT('Ctrl Pts',(62.5004397189015,-6.83522119344303,
40.0302263329211));
#167795=CARTESIAN_POINT('Ctrl Pts',(62.4884429377018,-6.84446844329974,
40.0127515884702));
#167796=CARTESIAN_POINT('Ctrl Pts',(62.4760404333281,-6.85402842900616,
39.9946858597657));
#167797=CARTESIAN_POINT('Ctrl Pts',(62.4633140048613,-6.86150157917988,
39.9757460620414));
#167798=CARTESIAN_POINT('Ctrl Pts',(62.4504583709314,-6.86692204703359,
39.9562444559034));
#167799=CARTESIAN_POINT('Ctrl Pts',(62.43784727821,-6.87223940618281,39.93711381135));
#167800=CARTESIAN_POINT('Ctrl Pts',(62.4251109433393,-6.87558122532823,
39.9174410654225));
#167801=CARTESIAN_POINT('Ctrl Pts',(62.4124375993731,-6.87693208138335,
39.8975196504));
#167802=CARTESIAN_POINT('Ctrl Pts',(62.4040419533072,-6.87782697616054,
39.8843224113677));
#167803=CARTESIAN_POINT('Ctrl Pts',(62.3956740599381,-6.87784715439598,
39.8710160447083));
#167804=CARTESIAN_POINT('Ctrl Pts',(62.3873926810691,-6.87697683366565,
39.8576902534424));
#167805=CARTESIAN_POINT('',(62.0330459552232,-6.8397366303026,39.2875012672119));
#167806=CARTESIAN_POINT('',(62.3873926810691,-6.87697683366565,39.8576902534424));
#167807=CARTESIAN_POINT('',(61.1105274371641,-12.6642893210142,39.2875012672119));
#167808=CARTESIAN_POINT('Origin',(5.53234440788222E-15,0.,39.2875012672119));
#167809=CARTESIAN_POINT('',(61.4590390555209,-12.7383709431251,39.8576902534424));
#167810=CARTESIAN_POINT('',(61.1105274371641,-12.6642893210142,39.2875012672119));
#167811=CARTESIAN_POINT('',(61.5816197022698,-13.0739701745325,40.1599502534424));
#167812=CARTESIAN_POINT('Ctrl Pts',(61.4590390555209,-12.7383709431251,
39.8576902534424));
#167813=CARTESIAN_POINT('Ctrl Pts',(61.4710760487545,-12.7409296199635,
39.8773836120357));
#167814=CARTESIAN_POINT('Ctrl Pts',(61.4826680729135,-12.7453875382442,
39.8969946442118));
#167815=CARTESIAN_POINT('Ctrl Pts',(61.4936637287782,-12.7516316867663,
39.916252528822));
#167816=CARTESIAN_POINT('Ctrl Pts',(61.5048803302315,-12.7580013045727,
39.9358973794034));
#167817=CARTESIAN_POINT('Ctrl Pts',(61.5154772731011,-12.7662298081581,
39.9551762199704));
#167818=CARTESIAN_POINT('Ctrl Pts',(61.5252915748192,-12.7762506512834,
39.97381520342));
#167819=CARTESIAN_POINT('Ctrl Pts',(61.5347245998124,-12.7858821937373,
39.9917300792592));
#167820=CARTESIAN_POINT('Ctrl Pts',(61.5434353195539,-12.7971700470085,
40.0090551158061));
#167821=CARTESIAN_POINT('Ctrl Pts',(61.5512651452145,-12.8100982055954,
40.0255394551466));
#167822=CARTESIAN_POINT('Ctrl Pts',(61.5572797455868,-12.8200291684063,
40.0382021526106));
#167823=CARTESIAN_POINT('Ctrl Pts',(61.5627743733232,-12.8309289078957,
40.0503687782102));
#167824=CARTESIAN_POINT('Ctrl Pts',(61.5676673859796,-12.8428059312035,
40.0619155352442));
#167825=CARTESIAN_POINT('Ctrl Pts',(61.5676802096931,-12.8428370587634,
40.0619457972351));
#167826=CARTESIAN_POINT('Ctrl Pts',(61.5676930289522,-12.8428681938091,
40.0619760547305));
#167827=CARTESIAN_POINT('Ctrl Pts',(61.5677058437553,-12.8428993363376,
40.0620063077269));
#167828=CARTESIAN_POINT('Ctrl Pts',(61.5690798512467,-12.8462384487037,
40.06525004417));
#167829=CARTESIAN_POINT('Ctrl Pts',(61.5704011254854,-12.8496624271213,
40.0684393223556));
#167830=CARTESIAN_POINT('Ctrl Pts',(61.5716678181342,-12.8531666956979,
40.0715697951759));
#167831=CARTESIAN_POINT('Ctrl Pts',(61.5787166747157,-12.8726671535591,
40.0889901646429));
#167832=CARTESIAN_POINT('Ctrl Pts',(61.5840799821732,-12.8946522063799,
40.1045963098259));
#167833=CARTESIAN_POINT('Ctrl Pts',(61.5874651029954,-12.9182844651727,
40.1176634650745));
#167834=CARTESIAN_POINT('Ctrl Pts',(61.5889843920985,-12.9288909501846,
40.1235281853075));
#167835=CARTESIAN_POINT('Ctrl Pts',(61.5901055263652,-12.9398294094013,
40.1288820140925));
#167836=CARTESIAN_POINT('Ctrl Pts',(61.5908034580838,-12.951025887472,40.1336621774101));
#167837=CARTESIAN_POINT('Ctrl Pts',(61.5911067697685,-12.9558917253992,
40.1357395717319));
#167838=CARTESIAN_POINT('Ctrl Pts',(61.5913300246961,-12.9608061353935,
40.1377083672884));
#167839=CARTESIAN_POINT('Ctrl Pts',(61.5914710890455,-12.9657629422643,
40.1395632548792));
#167840=CARTESIAN_POINT('Ctrl Pts',(61.5919648142682,-12.9831117663119,
40.146055361447));
#167841=CARTESIAN_POINT('Ctrl Pts',(61.5914517017518,-13.000979951431,40.151152097463));
#167842=CARTESIAN_POINT('Ctrl Pts',(61.5898402812905,-13.0191027399906,
40.1546258197409));
#167843=CARTESIAN_POINT('Ctrl Pts',(61.5890345710599,-13.0281641342704,
40.1563626808798));
#167844=CARTESIAN_POINT('Ctrl Pts',(61.5879542844384,-13.0372891795344,
40.1576937882008));
#167845=CARTESIAN_POINT('Ctrl Pts',(61.5865879953992,-13.046444782719,40.1585906813668));
#167846=CARTESIAN_POINT('Ctrl Pts',(61.5859048508796,-13.0510225843113,
40.1590391279498));
#167847=CARTESIAN_POINT('Ctrl Pts',(61.5851502058761,-13.0556080254095,
40.1593790209175));
#167848=CARTESIAN_POINT('Ctrl Pts',(61.5843226328192,-13.0601969695275,
40.1596068022931));
#167849=CARTESIAN_POINT('Ctrl Pts',(61.5834950597624,-13.0647859136456,
40.1598345836687));
#167850=CARTESIAN_POINT('Ctrl Pts',(61.5825945569831,-13.0693783604292,
40.1599502506864));
#167851=CARTESIAN_POINT('Ctrl Pts',(61.5816197022698,-13.0739701745325,
40.1599502534424));
#167852=CARTESIAN_POINT('',(61.5752716937451,-13.1038352065728,40.1599502534424));
#167853=CARTESIAN_POINT('Origin',(5.50318346416883E-15,5.72719669130613E-15,
40.1599502534424));
#167854=CARTESIAN_POINT('',(61.3267881959113,-13.3605623192487,39.8576902534424));
#167855=CARTESIAN_POINT('Ctrl Pts',(61.5752716937451,-13.1038352065728,
40.1599502534424));
#167856=CARTESIAN_POINT('Ctrl Pts',(61.5744762229326,-13.1075731191838,
40.1599502447858));
#167857=CARTESIAN_POINT('Ctrl Pts',(61.5736362456896,-13.1112908564312,
40.1598744685927));
#167858=CARTESIAN_POINT('Ctrl Pts',(61.5727532608743,-13.1149867645636,
40.1597246934279));
#167859=CARTESIAN_POINT('Ctrl Pts',(61.5676506979226,-13.1363445541695,
40.1588591777435));
#167860=CARTESIAN_POINT('Ctrl Pts',(61.5611131206557,-13.1569765024498,
40.1555254706021));
#167861=CARTESIAN_POINT('Ctrl Pts',(61.5534303645627,-13.1765564394372,
40.1500631826381));
#167862=CARTESIAN_POINT('Ctrl Pts',(61.5503317322969,-13.1844534784397,
40.1478601162481));
#167863=CARTESIAN_POINT('Ctrl Pts',(61.5470470005037,-13.192179815574,40.1453112228307));
#167864=CARTESIAN_POINT('Ctrl Pts',(61.5435957160157,-13.1997158239898,
40.1424401896328));
#167865=CARTESIAN_POINT('Ctrl Pts',(61.542322401576,-13.2024961535649,40.1413809526906));
#167866=CARTESIAN_POINT('Ctrl Pts',(61.5410263779726,-13.2052504481942,
40.1402777640512));
#167867=CARTESIAN_POINT('Ctrl Pts',(61.53970860908,-13.2079776587161,40.1391317641987));
#167868=CARTESIAN_POINT('Ctrl Pts',(61.5372377924063,-13.2130911784445,
40.1369830144753));
#167869=CARTESIAN_POINT('Ctrl Pts',(61.5346905274442,-13.2181094806066,
40.134683756585));
#167870=CARTESIAN_POINT('Ctrl Pts',(61.5320731679599,-13.223025649363,40.1322415082996));
#167871=CARTESIAN_POINT('Ctrl Pts',(61.5229124097647,-13.2402322400105,
40.1236936393009));
#167872=CARTESIAN_POINT('Ctrl Pts',(61.5128929892897,-13.2561876955039,
40.113394140767));
#167873=CARTESIAN_POINT('Ctrl Pts',(61.5022873490355,-13.2705955044753,
40.101665321223));
#167874=CARTESIAN_POINT('Ctrl Pts',(61.4969845289084,-13.277799408961,40.095800911451));
#167875=CARTESIAN_POINT('Ctrl Pts',(61.4915351548247,-13.284616402026,40.0895791707949));
#167876=CARTESIAN_POINT('Ctrl Pts',(61.4859732907799,-13.2910094216446,
40.0830403822907));
#167877=CARTESIAN_POINT('Ctrl Pts',(61.4831923587575,-13.2942059314539,
40.0797709880385));
#167878=CARTESIAN_POINT('Ctrl Pts',(61.4803833043595,-13.2972964479269,
40.0764223317514));
#167879=CARTESIAN_POINT('Ctrl Pts',(61.4775503861047,-13.3002763384266,
40.0729994484778));
#167880=CARTESIAN_POINT('Ctrl Pts',(61.4747174678498,-13.3032562289262,
40.0695765652042));
#167881=CARTESIAN_POINT('Ctrl Pts',(61.4718606611378,-13.3061253662367,
40.0660793733488));
#167882=CARTESIAN_POINT('Ctrl Pts',(61.4689842762858,-13.3088793779156,
40.0625130768817));
#167883=CARTESIAN_POINT('Ctrl Pts',(61.4689597467471,-13.3089028638675,
40.0624826638418));
#167884=CARTESIAN_POINT('Ctrl Pts',(61.4689352159238,-13.3089263414386,
40.0624522459912));
#167885=CARTESIAN_POINT('Ctrl Pts',(61.4689106838182,-13.3089498106269,
40.0624218233329));
#167886=CARTESIAN_POINT('Ctrl Pts',(61.4563817793396,-13.3209358677642,
40.04688452759));
#167887=CARTESIAN_POINT('Ctrl Pts',(61.4435806031496,-13.330852053932,40.030226332924));
#167888=CARTESIAN_POINT('Ctrl Pts',(61.4306829407567,-13.3387946412831,
40.0127515884748));
#167889=CARTESIAN_POINT('Ctrl Pts',(61.417349087986,-13.3470058416643,39.9946858597719));
#167890=CARTESIAN_POINT('Ctrl Pts',(61.4039112193236,-13.353107779129,39.9757460620493));
#167891=CARTESIAN_POINT('Ctrl Pts',(61.3905594167276,-13.357154773434,39.956244455913));
#167892=CARTESIAN_POINT('Ctrl Pts',(61.3774615935119,-13.3611247853915,
39.9371138113611));
#167893=CARTESIAN_POINT('Ctrl Pts',(61.3644457143973,-13.363116988191,39.917441065435));
#167894=CARTESIAN_POINT('Ctrl Pts',(61.3517005934285,-13.363135718947,39.897519650414));
#167895=CARTESIAN_POINT('Ctrl Pts',(61.3432573976113,-13.3631481274162,
39.884322411377));
#167896=CARTESIAN_POINT('Ctrl Pts',(61.3349332352346,-13.3622935120785,
39.8710160447129));
#167897=CARTESIAN_POINT('Ctrl Pts',(61.3267881959113,-13.3605623192487,
39.8576902534424));
#167898=CARTESIAN_POINT('',(60.9782752797348,-13.2864868028996,39.2875012672119));
#167899=CARTESIAN_POINT('',(61.3267881959113,-13.3605623192487,39.8576902534424));
#167900=CARTESIAN_POINT('',(59.4519788726607,-18.9827025415097,39.2875012672119));
#167901=CARTESIAN_POINT('Origin',(5.53234440788222E-15,0.,39.2875012672119));
#167902=CARTESIAN_POINT('',(59.7908376697911,-19.0928077206412,39.8576902534424));
#167903=CARTESIAN_POINT('',(59.4519788726608,-18.9827025415097,39.2875012672119));
#167904=CARTESIAN_POINT('',(59.8776671349985,-19.4393816709757,40.1599502534424));
#167905=CARTESIAN_POINT('Ctrl Pts',(59.7908376697911,-19.0928077206412,
39.8576902534424));
#167906=CARTESIAN_POINT('Ctrl Pts',(59.8025412685588,-19.0966105891853,
39.8773836120362));
#167907=CARTESIAN_POINT('Ctrl Pts',(59.8136038110496,-19.1022557829949,
39.8969946442128));
#167908=CARTESIAN_POINT('Ctrl Pts',(59.8238865403118,-19.1096150844286,
39.9162525288235));
#167909=CARTESIAN_POINT('Ctrl Pts',(59.8343758896881,-19.1171222629155,
39.9358973794055));
#167910=CARTESIAN_POINT('Ctrl Pts',(59.8440546685613,-19.1264133720511,
39.955176219973));
#167911=CARTESIAN_POINT('Ctrl Pts',(59.8527677431753,-19.1374051938264,
39.973815203423));
#167912=CARTESIAN_POINT('Ctrl Pts',(59.8611423227391,-19.14796999329,39.9917300792627));
#167913=CARTESIAN_POINT('Ctrl Pts',(59.8686254222905,-19.160106528669,40.00905511581));
#167914=CARTESIAN_POINT('Ctrl Pts',(59.8750609947969,-19.1737823050951,
40.0255394551508));
#167915=CARTESIAN_POINT('Ctrl Pts',(59.880004578277,-19.1842875619857,40.0382021526133));
#167916=CARTESIAN_POINT('Ctrl Pts',(59.8843297728483,-19.1957019365542,
40.0503687782115));
#167917=CARTESIAN_POINT('Ctrl Pts',(59.8879544940744,-19.2080253553779,
40.0619155352442));
#167918=CARTESIAN_POINT('Ctrl Pts',(59.8879639938223,-19.2080576528609,
40.0619457972351));
#167919=CARTESIAN_POINT('Ctrl Pts',(59.8879734883577,-19.208089957323,40.0619760547305));
#167920=CARTESIAN_POINT('Ctrl Pts',(59.8879829776793,-19.2081222687611,
40.0620063077269));
#167921=CARTESIAN_POINT('Ctrl Pts',(59.8890004259296,-19.2115867120118,
40.06525004417));
#167922=CARTESIAN_POINT('Ctrl Pts',(59.8899565588875,-19.2151300442832,
40.0684393223556));
#167923=CARTESIAN_POINT('Ctrl Pts',(59.8908500166522,-19.2187475215459,
40.0715697951759));
#167924=CARTESIAN_POINT('Ctrl Pts',(59.8958219059664,-19.2388779600041,
40.0889901646423));
#167925=CARTESIAN_POINT('Ctrl Pts',(59.8988577688783,-19.261303194691,40.1045963098248));
#167926=CARTESIAN_POINT('Ctrl Pts',(59.8997541019594,-19.285159834974,40.1176634650732));
#167927=CARTESIAN_POINT('Ctrl Pts',(59.9001563886589,-19.2958670255072,
40.1235281853067));
#167928=CARTESIAN_POINT('Ctrl Pts',(59.9001280009024,-19.3068627531426,
40.1288820140922));
#167929=CARTESIAN_POINT('Ctrl Pts',(59.8996517586312,-19.3180708494659,
40.1336621774101));
#167930=CARTESIAN_POINT('Ctrl Pts',(59.8994447901818,-19.322941736528,40.1357395717319));
#167931=CARTESIAN_POINT('Ctrl Pts',(59.8991531263709,-19.3278525613647,
40.1377083672884));
#167932=CARTESIAN_POINT('Ctrl Pts',(59.8987752905501,-19.3327969595684,
40.1395632548792));
#167933=CARTESIAN_POINT('Ctrl Pts',(59.8974528651773,-19.3501023532815,
40.146055361447));
#167934=CARTESIAN_POINT('Ctrl Pts',(59.895074829613,-19.3678190197501,40.1511520974629));
#167935=CARTESIAN_POINT('Ctrl Pts',(59.8915778894434,-19.3856740904733,
40.1546258197408));
#167936=CARTESIAN_POINT('Ctrl Pts',(59.8898294193586,-19.3946016258349,
40.1563626808798));
#167937=CARTESIAN_POINT('Ctrl Pts',(59.8878012237015,-19.4035637624457,
40.1576937882008));
#167938=CARTESIAN_POINT('Ctrl Pts',(59.8854853982054,-19.4125263941844,
40.1585906813668));
#167939=CARTESIAN_POINT('Ctrl Pts',(59.8843274854574,-19.4170077100538,
40.1590391279498));
#167940=CARTESIAN_POINT('Ctrl Pts',(59.8830976653668,-19.4214891497433,
40.1593790209175));
#167941=CARTESIAN_POINT('Ctrl Pts',(59.881794950565,-19.4259664502055,40.1596068022931));
#167942=CARTESIAN_POINT('Ctrl Pts',(59.8804922357633,-19.4304437506676,
40.1598345836687));
#167943=CARTESIAN_POINT('Ctrl Pts',(59.8791166246276,-19.4349169113756,
40.1599502506865));
#167944=CARTESIAN_POINT('Ctrl Pts',(59.8776671349985,-19.4393816709757,
40.1599502534424));
#167945=CARTESIAN_POINT('',(59.8682321556242,-19.4684195516697,40.1599502534424));
#167946=CARTESIAN_POINT('Origin',(5.50739376141089E-15,5.74290973452844E-15,
40.1599502534424));
#167947=CARTESIAN_POINT('',(59.5942745858235,-19.6977666881846,39.8576902534424));
#167948=CARTESIAN_POINT('Ctrl Pts',(59.8682321556242,-19.4684195516697,
40.1599502534424));
#167949=CARTESIAN_POINT('Ctrl Pts',(59.8670503242229,-19.4720538382627,
40.1599502447858));
#167950=CARTESIAN_POINT('Ctrl Pts',(59.8658263391019,-19.4756634078261,
40.1598744685927));
#167951=CARTESIAN_POINT('Ctrl Pts',(59.8645618637724,-19.4792467723412,
40.1597246934279));
#167952=CARTESIAN_POINT('Ctrl Pts',(59.8572547562668,-19.4999541986804,
40.1588591777433));
#167953=CARTESIAN_POINT('Ctrl Pts',(59.8485963666826,-19.5197897600872,
40.1555254706009));
#167954=CARTESIAN_POINT('Ctrl Pts',(59.8389090368052,-19.5384593694458,
40.1500631826353));
#167955=CARTESIAN_POINT('Ctrl Pts',(59.8350019138213,-19.5459892523701,
40.147860116246));
#167956=CARTESIAN_POINT('Ctrl Pts',(59.8309275539868,-19.5533299158514,
40.1453112228295));
#167957=CARTESIAN_POINT('Ctrl Pts',(59.8267074486193,-19.5604638837579,
40.1424401896328));
#167958=CARTESIAN_POINT('Ctrl Pts',(59.8251504859514,-19.563095884795,40.1413809526905));
#167959=CARTESIAN_POINT('Ctrl Pts',(59.8235736599159,-19.5656996197545,
40.1402777640511));
#167960=CARTESIAN_POINT('Ctrl Pts',(59.8219780387743,-19.5682741459745,
40.1391317641986));
#167961=CARTESIAN_POINT('Ctrl Pts',(59.8189862491338,-19.573101382637,40.1369830144753));
#167962=CARTESIAN_POINT('Ctrl Pts',(59.8159283829425,-19.5778259323227,
40.1346837565849));
#167963=CARTESIAN_POINT('Ctrl Pts',(59.812811482062,-19.5824415812275,40.1322415082995));
#167964=CARTESIAN_POINT('Ctrl Pts',(59.8019023289803,-19.5985963523946,
40.1236936393008));
#167965=CARTESIAN_POINT('Ctrl Pts',(59.7902699966956,-19.6134170876082,
40.113394140767));
#167966=CARTESIAN_POINT('Ctrl Pts',(59.7782164291175,-19.6266373778168,
40.101665321223));
#167967=CARTESIAN_POINT('Ctrl Pts',(59.7721896453285,-19.6332475229211,
40.095800911451));
#167968=CARTESIAN_POINT('Ctrl Pts',(59.7660575536771,-19.6394575570861,
40.0895791707949));
#167969=CARTESIAN_POINT('Ctrl Pts',(59.7598579055891,-19.6452341819728,
40.0830403822906));
#167970=CARTESIAN_POINT('Ctrl Pts',(59.7567580815451,-19.6481224944161,
40.0797709880385));
#167971=CARTESIAN_POINT('Ctrl Pts',(59.7536413685033,-19.6509024545771,
40.0764223317514));
#167972=CARTESIAN_POINT('Ctrl Pts',(59.7505124858965,-19.6535699003331,
40.0729994484778));
#167973=CARTESIAN_POINT('Ctrl Pts',(59.7473836032896,-19.656237346089,40.0695765652042));
#167974=CARTESIAN_POINT('Ctrl Pts',(59.7442425399497,-19.6587921483496,
40.0660793733488));
#167975=CARTESIAN_POINT('Ctrl Pts',(59.7410940396263,-19.6612304091761,
40.0625130768817));
#167976=CARTESIAN_POINT('Ctrl Pts',(59.7410671895125,-19.6612512024345,
40.0624826638418));
#167977=CARTESIAN_POINT('Ctrl Pts',(59.7410403389972,-19.6612719872237,
40.0624522459912));
#167978=CARTESIAN_POINT('Ctrl Pts',(59.7410134880829,-19.6612927635421,
40.0624218233329));
#167979=CARTESIAN_POINT('Ctrl Pts',(59.7273003341212,-19.6719035326722,
40.0468845275906));
#167980=CARTESIAN_POINT('Ctrl Pts',(59.7135327604127,-19.6804273096593,
40.0302263329252));
#167981=CARTESIAN_POINT('Ctrl Pts',(59.6998755263142,-19.6869782138561,
40.0127515884767));
#167982=CARTESIAN_POINT('Ctrl Pts',(59.6857564136272,-19.6937506652829,
39.9946858597746));
#167983=CARTESIAN_POINT('Ctrl Pts',(59.6717543328698,-19.6984145359349,
39.9757460620528));
#167984=CARTESIAN_POINT('Ctrl Pts',(59.6580526467503,-19.7010437169746,
39.9562444559175));
#167985=CARTESIAN_POINT('Ctrl Pts',(59.6446115955321,-19.7036228854586,
39.9371138113664));
#167986=CARTESIAN_POINT('Ctrl Pts',(59.6314587768685,-19.7042436449211,
39.9174410654413));
#167987=CARTESIAN_POINT('Ctrl Pts',(59.6187815171093,-19.7029300451595,
39.8975196504211));
#167988=CARTESIAN_POINT('Ctrl Pts',(59.6103832769623,-19.7020598313701,
39.8843224113819));
#167989=CARTESIAN_POINT('Ctrl Pts',(59.6021940468446,-19.7003397858032,
39.8710160447154));
#167990=CARTESIAN_POINT('Ctrl Pts',(59.5942745858236,-19.6977666881846,
39.8576902534424));
#167991=CARTESIAN_POINT('',(59.2554138597571,-19.5876674457079,39.2875012672119));
#167992=CARTESIAN_POINT('',(59.5942745858236,-19.6977666881846,39.8576902534424));
#167993=CARTESIAN_POINT('',(57.1420619865021,-25.0931373005746,39.2875012672119));
#167994=CARTESIAN_POINT('Origin',(5.53234440788222E-15,0.,39.2875012672119));
#167995=CARTESIAN_POINT('',(57.467555354514,-25.2380597013431,39.8576902534424));
#167996=CARTESIAN_POINT('',(57.1420619865021,-25.0931373005746,39.2875012672119));
#167997=CARTESIAN_POINT('',(57.5176823163888,-25.5918112338795,40.1599502534424));
#167998=CARTESIAN_POINT('Ctrl Pts',(57.467555354514,-25.2380597013431,39.8576902534424));
#167999=CARTESIAN_POINT('Ctrl Pts',(57.4787973317376,-25.2430650965691,
39.8773836120353));
#168000=CARTESIAN_POINT('Ctrl Pts',(57.489209189029,-25.2498357159823,39.896994644211));
#168001=CARTESIAN_POINT('Ctrl Pts',(57.4986663319544,-25.2582295402801,
39.9162525288208));
#168002=CARTESIAN_POINT('Ctrl Pts',(57.5083135057462,-25.2667920292282,
39.9358973794019));
#168003=CARTESIAN_POINT('Ctrl Pts',(57.5169680778957,-25.2770439485771,
39.9551762199685));
#168004=CARTESIAN_POINT('Ctrl Pts',(57.5244844631365,-25.2888863203014,
39.9738152034178));
#168005=CARTESIAN_POINT('Ctrl Pts',(57.5317088436245,-25.3002686266197,
39.9917300792568));
#168006=CARTESIAN_POINT('Ctrl Pts',(57.537882336581,-25.3131208736838,40.0090551158036));
#168007=CARTESIAN_POINT('Ctrl Pts',(57.5428531464542,-25.3273944332791,
40.025539455144));
#168008=CARTESIAN_POINT('Ctrl Pts',(57.5466715501087,-25.3383588864591,
40.0382021526089));
#168009=CARTESIAN_POINT('Ctrl Pts',(57.5497799237794,-25.3501628378332,
40.0503687782094));
#168010=CARTESIAN_POINT('Ctrl Pts',(57.552096640372,-25.362797634221,40.0619155352442));
#168011=CARTESIAN_POINT('Ctrl Pts',(57.552102712073,-25.3628307477691,40.0619457972351));
#168012=CARTESIAN_POINT('Ctrl Pts',(57.5521087778605,-25.3628638677132,
40.0619760547304));
#168013=CARTESIAN_POINT('Ctrl Pts',(57.5521148377337,-25.3628969940501,
40.0620063077269));
#168014=CARTESIAN_POINT('Ctrl Pts',(57.552764579367,-25.3664488110202,40.06525004417));
#168015=CARTESIAN_POINT('Ctrl Pts',(57.5533450954513,-25.3700726756554,
40.0684393223556));
#168016=CARTESIAN_POINT('Ctrl Pts',(57.5538555294217,-25.3737637277663,
40.0715697951758));
#168017=CARTESIAN_POINT('Ctrl Pts',(57.5566959784089,-25.3943035935241,
40.0889901646408));
#168018=CARTESIAN_POINT('Ctrl Pts',(57.5573711352259,-25.4169233145116,
40.104596309822));
#168019=CARTESIAN_POINT('Ctrl Pts',(57.5557688601537,-25.4407429579403,
40.1176634650697));
#168020=CARTESIAN_POINT('Ctrl Pts',(57.5550497369122,-25.4514335437759,
40.1235281853045));
#168021=CARTESIAN_POINT('Ctrl Pts',(57.5538721381544,-25.4623660683384,
40.1288820140912));
#168022=CARTESIAN_POINT('Ctrl Pts',(57.5522269397031,-25.4734629846667,
40.1336621774101));
#168023=CARTESIAN_POINT('Ctrl Pts',(57.5515119587091,-25.4782855544059,
40.1357395717319));
#168024=CARTESIAN_POINT('Ctrl Pts',(57.5507085716896,-25.4831389900603,
40.1377083672884));
#168025=CARTESIAN_POINT('Ctrl Pts',(57.5498159753469,-25.4880168077357,
40.1395632548792));
#168026=CARTESIAN_POINT('Ctrl Pts',(57.5466918881476,-25.5050891695993,
40.146055361447));
#168027=CARTESIAN_POINT('Ctrl Pts',(57.5424749837907,-25.5224602099121,
40.1511520974629));
#168028=CARTESIAN_POINT('Ctrl Pts',(57.5371308371211,-25.5398519389076,
40.1546258197408));
#168029=CARTESIAN_POINT('Ctrl Pts',(57.5344587637862,-25.5485478034053,
40.1563626808798));
#168030=CARTESIAN_POINT('Ctrl Pts',(57.5315048804296,-25.5572488403188,
40.1576937882008));
#168031=CARTESIAN_POINT('Ctrl Pts',(57.5282648911454,-25.5659203041428,
40.1585906813668));
#168032=CARTESIAN_POINT('Ctrl Pts',(57.5266448965033,-25.5702560360549,
40.1590391279498));
#168033=CARTESIAN_POINT('Ctrl Pts',(57.5249533754919,-25.5745843747447,
40.1593790209175));
#168034=CARTESIAN_POINT('Ctrl Pts',(57.5231897917613,-25.5789009773101,
40.1596068022931));
#168035=CARTESIAN_POINT('Ctrl Pts',(57.5214262080306,-25.5832175798756,
40.1598345836687));
#168036=CARTESIAN_POINT('Ctrl Pts',(57.5195905600219,-25.587522445623,40.1599502506865));
#168037=CARTESIAN_POINT('Ctrl Pts',(57.5176823163888,-25.5918112338795,
40.1599502534424));
#168038=CARTESIAN_POINT('',(57.5052637377732,-25.6197038181298,40.1599502534424));
#168039=CARTESIAN_POINT('Origin',(5.5132234544654E-15,5.75809660415529E-15,
40.1599502534424));
#168040=CARTESIAN_POINT('',(57.2088336324698,-25.8191582032621,39.8576902534424));
#168041=CARTESIAN_POINT('Ctrl Pts',(57.5052637377732,-25.6197038181299,
40.1599502534424));
#168042=CARTESIAN_POINT('Ctrl Pts',(57.5037084941754,-25.6231946607004,
40.1599502447858));
#168043=CARTESIAN_POINT('Ctrl Pts',(57.5021139114133,-25.6266565153803,
40.1598744685927));
#168044=CARTESIAN_POINT('Ctrl Pts',(57.5004817994259,-25.6300880761866,
40.1597246934279));
#168045=CARTESIAN_POINT('Ctrl Pts',(57.4910502055677,-25.6499182643563,
40.1588591777434));
#168046=CARTESIAN_POINT('Ctrl Pts',(57.4803658667974,-25.6687401163222,
40.1555254706019));
#168047=CARTESIAN_POINT('Ctrl Pts',(57.4687800995525,-25.6862948498998,
40.1500631826377));
#168048=CARTESIAN_POINT('Ctrl Pts',(57.4641072931049,-25.6933750777789,
40.1478601162478));
#168049=CARTESIAN_POINT('Ctrl Pts',(57.4592879447652,-25.7002496417679,
40.1453112228305));
#168050=CARTESIAN_POINT('Ctrl Pts',(57.4543452548725,-25.7069034079251,
40.1424401896328));
#168051=CARTESIAN_POINT('Ctrl Pts',(57.4525217023852,-25.7093582436701,
40.1413809526906));
#168052=CARTESIAN_POINT('Ctrl Pts',(57.4506813499537,-25.7117828918948,
40.1402777640512));
#168053=CARTESIAN_POINT('Ctrl Pts',(57.4488253585223,-25.7141765267649,
40.1391317641987));
#168054=CARTESIAN_POINT('Ctrl Pts',(57.4453453745883,-25.7186645921463,
40.1369830144753));
#168055=CARTESIAN_POINT('Ctrl Pts',(57.4418104097897,-25.7230436262006,
40.134683756585));
#168056=CARTESIAN_POINT('Ctrl Pts',(57.4382281169313,-25.7273081852386,
40.1322415082996));
#168057=CARTESIAN_POINT('Ctrl Pts',(57.4256900919271,-25.7422341418718,
40.1236936393009));
#168058=CARTESIAN_POINT('Ctrl Pts',(57.4125722940993,-25.7557577777292,
40.113394140767));
#168059=CARTESIAN_POINT('Ctrl Pts',(57.3992028606062,-25.767645704909,40.101665321223));
#168060=CARTESIAN_POINT('Ctrl Pts',(57.3925181438596,-25.7735896684989,
40.095800911451));
#168061=CARTESIAN_POINT('Ctrl Pts',(57.3857705191197,-25.7791247053301,
40.0895791707949));
#168062=CARTESIAN_POINT('Ctrl Pts',(57.3790010116303,-25.7842216455737,
40.0830403822906));
#168063=CARTESIAN_POINT('Ctrl Pts',(57.3756162578857,-25.7867701156956,
40.0797709880385));
#168064=CARTESIAN_POINT('Ctrl Pts',(57.3722260335605,-25.7892090617192,
40.0764223317514));
#168065=CARTESIAN_POINT('Ctrl Pts',(57.3688354672942,-25.7915348376376,
40.0729994484778));
#168066=CARTESIAN_POINT('Ctrl Pts',(57.3654449010279,-25.793860613556,40.0695765652042));
#168067=CARTESIAN_POINT('Ctrl Pts',(57.3620539952074,-25.7960730898185,
40.0660793733488));
#168068=CARTESIAN_POINT('Ctrl Pts',(57.358667875041,-25.7981688856967,40.0625130768817));
#168069=CARTESIAN_POINT('Ctrl Pts',(57.3586389985276,-25.7981867584462,
40.0624826638418));
#168070=CARTESIAN_POINT('Ctrl Pts',(57.3586101225001,-25.7982046227311,
40.0624522459912));
#168071=CARTESIAN_POINT('Ctrl Pts',(57.3585812469612,-25.7982224785499,
40.0624218233329));
#168072=CARTESIAN_POINT('Ctrl Pts',(57.3438340877008,-25.8073417058662,
40.0468845275908));
#168073=CARTESIAN_POINT('Ctrl Pts',(57.3292509568922,-25.8143796853882,
40.0302263329259));
#168074=CARTESIAN_POINT('Ctrl Pts',(57.3149837826027,-25.8194671333536,
40.0127515884777));
#168075=CARTESIAN_POINT('Ctrl Pts',(57.3002341019524,-25.8247266354309,
39.9946858597759));
#168076=CARTESIAN_POINT('Ctrl Pts',(57.2858212188265,-25.8279013409274,
39.9757460620546));
#168077=CARTESIAN_POINT('Ctrl Pts',(57.2719197677237,-25.8290839028441,
39.9562444559196));
#168078=CARTESIAN_POINT('Ctrl Pts',(57.2582827514725,-25.8302439699449,
39.9371138113688));
#168079=CARTESIAN_POINT('Ctrl Pts',(57.2451370982931,-25.8294864848997,
39.9174410654439));
#168080=CARTESIAN_POINT('Ctrl Pts',(57.2326665944538,-25.8268549466943,
39.897519650424));
#168081=CARTESIAN_POINT('Ctrl Pts',(57.2244053228545,-25.8251116448903,
39.8843224113838));
#168082=CARTESIAN_POINT('Ctrl Pts',(57.2164407479154,-25.8225450142734,
39.8710160447163));
#168083=CARTESIAN_POINT('Ctrl Pts',(57.2088336324698,-25.8191582032621,
39.8576902534424));
#168084=CARTESIAN_POINT('',(56.8833377255394,-25.6742415049981,39.2875012672119));
#168085=CARTESIAN_POINT('',(57.2088336324698,-25.8191582032621,39.8576902534424));
#168086=CARTESIAN_POINT('',(54.2060847114741,-30.9286463962979,39.2875012672119));
#168087=CARTESIAN_POINT('Origin',(5.53234440788222E-15,0.,39.2875012672119));
#168088=CARTESIAN_POINT('',(54.5146464769137,-31.1067982185536,39.8576902534424));
#168089=CARTESIAN_POINT('',(54.2060847114741,-30.9286463962979,39.2875012672119));
#168090=CARTESIAN_POINT('',(54.5275217339719,-31.4638515574741,40.1599502534424));
#168091=CARTESIAN_POINT('Ctrl Pts',(54.5146464769138,-31.1067982185536,
39.8576902534424));
#168092=CARTESIAN_POINT('Ctrl Pts',(54.5253036631384,-31.1129513003039,
39.8773836120346));
#168093=CARTESIAN_POINT('Ctrl Pts',(54.5349507607431,-31.1207731649977,
39.8969946442096));
#168094=CARTESIAN_POINT('Ctrl Pts',(54.543478702895,-31.1301095476642,39.9162525288187));
#168095=CARTESIAN_POINT('Ctrl Pts',(54.5521780046476,-31.1396335346527,
39.935897379399));
#168096=CARTESIAN_POINT('Ctrl Pts',(54.5597135487701,-31.1507339420411,
39.9551762199648));
#168097=CARTESIAN_POINT('Ctrl Pts',(54.5659508935483,-31.1632971162118,
39.9738152034134));
#168098=CARTESIAN_POINT('Ctrl Pts',(54.5719459231361,-31.1753722224548,
39.9917300792516));
#168099=CARTESIAN_POINT('Ctrl Pts',(54.5767421714171,-31.1887993692954,
40.0090551157976));
#168100=CARTESIAN_POINT('Ctrl Pts',(54.580193757424,-31.2035143279539,40.0255394551374));
#168101=CARTESIAN_POINT('Ctrl Pts',(54.582845146023,-31.21481784858,40.0382021526047));
#168102=CARTESIAN_POINT('Ctrl Pts',(54.5847026428005,-31.2268820501984,
40.0503687782074));
#168103=CARTESIAN_POINT('Ctrl Pts',(54.5856859723272,-31.2396897946771,
40.0619155352442));
#168104=CARTESIAN_POINT('Ctrl Pts',(54.5856885494585,-31.2397233614912,
40.0619457972351));
#168105=CARTESIAN_POINT('Ctrl Pts',(54.5856911200402,-31.2397569340482,
40.0619760547304));
#168106=CARTESIAN_POINT('Ctrl Pts',(54.5856936840716,-31.2397905123448,
40.0620063077269));
#168107=CARTESIAN_POINT('Ctrl Pts',(54.5859686003825,-31.2433907885844,
40.06525004417));
#168108=CARTESIAN_POINT('Ctrl Pts',(54.5861671393376,-31.2470554817642,
40.0684393223556));
#168109=CARTESIAN_POINT('Ctrl Pts',(54.5862889570923,-31.2507796687839,
40.0715697951759));
#168110=CARTESIAN_POINT('Ctrl Pts',(54.5869668451994,-31.2715039227768,
40.0889901646418));
#168111=CARTESIAN_POINT('Ctrl Pts',(54.5852738987621,-31.294070303672,40.1045963098239));
#168112=CARTESIAN_POINT('Ctrl Pts',(54.5811905703967,-31.3175919772521,
40.117663465072));
#168113=CARTESIAN_POINT('Ctrl Pts',(54.5793579160789,-31.3281488300913,
40.123528185306));
#168114=CARTESIAN_POINT('Ctrl Pts',(54.5770440083384,-31.3388983725505,
40.1288820140919));
#168115=CARTESIAN_POINT('Ctrl Pts',(54.5742478788459,-31.3497625287428,
40.1336621774101));
#168116=CARTESIAN_POINT('Ctrl Pts',(54.5730327187888,-31.3544839440758,
40.1357395717319));
#168117=CARTESIAN_POINT('Ctrl Pts',(54.5717264106368,-31.3592268152913,
40.1377083672884));
#168118=CARTESIAN_POINT('Ctrl Pts',(54.5703288332446,-31.363984610047,40.1395632548792));
#168119=CARTESIAN_POINT('Ctrl Pts',(54.5654373123719,-31.380636891692,40.146055361447));
#168120=CARTESIAN_POINT('Ctrl Pts',(54.559427740509,-31.3974719850962,40.1511520974629));
#168121=CARTESIAN_POINT('Ctrl Pts',(54.5522949389285,-31.4142098249417,
40.1546258197408));
#168122=CARTESIAN_POINT('Ctrl Pts',(54.5487285381383,-31.4225787448644,
40.1563626808798));
#168123=CARTESIAN_POINT('Ctrl Pts',(54.5448813304464,-31.4309233516993,
40.1576937882008));
#168124=CARTESIAN_POINT('Ctrl Pts',(54.5407526753747,-31.4392086412363,
40.1585906813668));
#168125=CARTESIAN_POINT('Ctrl Pts',(54.5386883478389,-31.4433512860048,
40.1590391279498));
#168126=CARTESIAN_POINT('Ctrl Pts',(54.5365536585648,-31.4474791015105,
40.1593790209175));
#168127=CARTESIAN_POINT('Ctrl Pts',(54.5343485280976,-31.4515877125783,
40.1596068022931));
#168128=CARTESIAN_POINT('Ctrl Pts',(54.5321433976304,-31.455696323646,40.1598345836687));
#168129=CARTESIAN_POINT('Ctrl Pts',(54.5298678244924,-31.459785729423,40.1599502506864));
#168130=CARTESIAN_POINT('Ctrl Pts',(54.5275217339719,-31.4638515574741,
40.1599502534424));
#168131=CARTESIAN_POINT('',(54.5122556166611,-31.4902932482908,40.1599502534424));
#168132=CARTESIAN_POINT('Origin',(5.52060867199534E-15,5.77259090966498E-15,
40.1599502534424));
#168133=CARTESIAN_POINT('',(54.1966007261207,-31.6576696180585,39.8576902534424));
#168134=CARTESIAN_POINT('Ctrl Pts',(54.512255616661,-31.4902932482908,40.1599502534424));
#168135=CARTESIAN_POINT('Ctrl Pts',(54.510344000441,-31.4936024004372,40.1599502447858));
#168136=CARTESIAN_POINT('Ctrl Pts',(54.5083962906204,-31.4968786114293,
40.1598744685927));
#168137=CARTESIAN_POINT('Ctrl Pts',(54.5064144237356,-31.5001207716285,
40.1597246934279));
#168138=CARTESIAN_POINT('Ctrl Pts',(54.4949616780398,-31.5188564579403,
40.1588591777435));
#168139=CARTESIAN_POINT('Ctrl Pts',(54.4823684499334,-31.5364583843189,
40.1555254706019));
#168140=CARTESIAN_POINT('Ctrl Pts',(54.4690111814099,-31.5527059087832,
40.1500631826378));
#168141=CARTESIAN_POINT('Ctrl Pts',(54.4636238877451,-31.5592589091562,
40.1478601162479));
#168142=CARTESIAN_POINT('Ctrl Pts',(54.4581123526903,-31.5655920544886,
40.1453112228306));
#168143=CARTESIAN_POINT('Ctrl Pts',(54.4525012314185,-31.5716927188399,
40.1424401896328));
#168144=CARTESIAN_POINT('Ctrl Pts',(54.4504310683346,-31.5739434935987,
40.1413809526906));
#168145=CARTESIAN_POINT('Ctrl Pts',(54.4483473527934,-31.5761624901351,
40.1402777640511));
#168146=CARTESIAN_POINT('Ctrl Pts',(54.4462513257026,-31.5783490084907,
40.1391317641987));
#168147=CARTESIAN_POINT('Ctrl Pts',(54.4423212749073,-31.5824487304076,
40.1369830144753));
#168148=CARTESIAN_POINT('Ctrl Pts',(54.4383479413154,-31.5864342712171,
40.1346837565849));
#168149=CARTESIAN_POINT('Ctrl Pts',(54.4343395048294,-31.590301016987,40.1322415082996));
#168150=CARTESIAN_POINT('Ctrl Pts',(54.4203099771284,-31.6038346271819,
40.1236936393008));
#168151=CARTESIAN_POINT('Ctrl Pts',(54.4058504350957,-31.6159129958987,
40.113394140767));
#168152=CARTESIAN_POINT('Ctrl Pts',(54.3913116139986,-31.6263383134317,
40.101665321223));
#168153=CARTESIAN_POINT('Ctrl Pts',(54.38404220345,-31.6315509721983,40.095800911451));
#168154=CARTESIAN_POINT('Ctrl Pts',(54.3767529740103,-31.6363503686737,
40.0895791707949));
#168155=CARTESIAN_POINT('Ctrl Pts',(54.3694877752603,-31.6407117811305,
40.0830403822906));
#168156=CARTESIAN_POINT('Ctrl Pts',(54.3658551758852,-31.6428924873589,
40.0797709880385));
#168157=CARTESIAN_POINT('Ctrl Pts',(54.3622285842838,-31.6449636976422,
40.0764223317514));
#168158=CARTESIAN_POINT('Ctrl Pts',(54.3586134821116,-31.6469223220353,
40.0729994484778));
#168159=CARTESIAN_POINT('Ctrl Pts',(54.3549983799394,-31.6488809464285,
40.0695765652042));
#168160=CARTESIAN_POINT('Ctrl Pts',(54.3513947831121,-31.65072685634,40.0660793733488));
#168161=CARTESIAN_POINT('Ctrl Pts',(54.3478081421437,-31.6524572252917,
40.0625130768817));
#168162=CARTESIAN_POINT('Ctrl Pts',(54.3477775556079,-31.6524719817149,
40.0624826638418));
#168163=CARTESIAN_POINT('Ctrl Pts',(54.34774697044,-31.6524867297705,40.0624522459912));
#168164=CARTESIAN_POINT('Ctrl Pts',(54.3477163866431,-31.6525014694575,
40.0624218233329));
#168165=CARTESIAN_POINT('Ctrl Pts',(54.3320967950454,-31.6600292427979,
40.0468845275897));
#168166=CARTESIAN_POINT('Ctrl Pts',(54.3168578829681,-31.665504315279,40.0302263329234));
#168167=CARTESIAN_POINT('Ctrl Pts',(54.3021370826333,-31.6690725678684,
40.0127515884738));
#168168=CARTESIAN_POINT('Ctrl Pts',(54.2869184346062,-31.672761496391,39.9946858597706));
#168169=CARTESIAN_POINT('Ctrl Pts',(54.2722526596743,-31.6744122539939,
39.9757460620476));
#168170=CARTESIAN_POINT('Ctrl Pts',(54.2583037507945,-31.6741352403912,
39.9562444559111));
#168171=CARTESIAN_POINT('Ctrl Pts',(54.2446201795132,-31.6738634961701,
39.9371138113589));
#168172=CARTESIAN_POINT('Ctrl Pts',(54.2316257183445,-31.671736065781,39.9174410654326));
#168173=CARTESIAN_POINT('Ctrl Pts',(54.2194985998743,-31.6678154208136,
39.8975196504113));
#168174=CARTESIAN_POINT('Ctrl Pts',(54.2114648090467,-31.6652181309748,
39.8843224113753));
#168175=CARTESIAN_POINT('Ctrl Pts',(54.2038121508392,-31.6618330358508,
39.871016044712));
#168176=CARTESIAN_POINT('Ctrl Pts',(54.1966007261207,-31.6576696180585,
39.8576902534424));
#168177=CARTESIAN_POINT('',(53.888035839597,-31.479523201679,39.2875012672119));
#168178=CARTESIAN_POINT('',(54.1966007261207,-31.6576696180585,39.8576902534424));
#168179=CARTESIAN_POINT('',(50.6762142289948,-36.4252947698679,39.2875012672119));
#168180=CARTESIAN_POINT('Origin',(5.53234440788222E-15,0.,39.2875012672119));
#168181=CARTESIAN_POINT('',(50.9644637245892,-36.6347241449655,39.8576902534424));
#168182=CARTESIAN_POINT('',(50.6762142289948,-36.4252947698679,39.2875012672119));
#168183=CARTESIAN_POINT('',(50.9399462128201,-36.9911673391708,40.1599502534424));
#168184=CARTESIAN_POINT('Ctrl Pts',(50.9644637245892,-36.6347241449655,
39.8576902534424));
#168185=CARTESIAN_POINT('Ctrl Pts',(50.9744193574531,-36.641957498789,39.8773836120347));
#168186=CARTESIAN_POINT('Ctrl Pts',(50.9831959997515,-36.6507449107773,
39.8969946442099));
#168187=CARTESIAN_POINT('Ctrl Pts',(50.9907013072115,-36.6609215604507,
39.9162525288192));
#168188=CARTESIAN_POINT('Ctrl Pts',(50.9983574255548,-36.6713026986859,
39.9358973793998));
#168189=CARTESIAN_POINT('Ctrl Pts',(51.0046913806523,-36.6831299757284,
39.9551762199659));
#168190=CARTESIAN_POINT('Ctrl Pts',(51.0095813473133,-36.6962763075813,
39.9738152034147));
#168191=CARTESIAN_POINT('Ctrl Pts',(51.0142813432023,-36.7089119163592,
39.9917300792533));
#168192=CARTESIAN_POINT('Ctrl Pts',(51.0176477981081,-36.7227668523472,
40.0090551157996));
#168193=CARTESIAN_POINT('Ctrl Pts',(51.01954234395,-36.7377619899041,40.0255394551396));
#168194=CARTESIAN_POINT('Ctrl Pts',(51.0209976683241,-36.7492807342367,
40.0382021526061));
#168195=CARTESIAN_POINT('Ctrl Pts',(51.021583937084,-36.7614730081793,40.0503687782081));
#168196=CARTESIAN_POINT('Ctrl Pts',(51.0212231059804,-36.7743133764172,
40.0619155352442));
#168197=CARTESIAN_POINT('Ctrl Pts',(51.0212221603065,-36.7743470287324,
40.0619457972351));
#168198=CARTESIAN_POINT('Ctrl Pts',(51.0212212075184,-36.7743806860744,
40.0619760547304));
#168199=CARTESIAN_POINT('Ctrl Pts',(51.021220247616,-36.7744143484398,40.0620063077269));
#168200=CARTESIAN_POINT('Ctrl Pts',(51.021117326564,-36.778023638569,40.06525004417));
#168201=CARTESIAN_POINT('Ctrl Pts',(51.0209317131555,-36.7816890091479,
40.0684393223556));
#168202=CARTESIAN_POINT('Ctrl Pts',(51.0206635800337,-36.7854055281042,
40.0715697951759));
#168203=CARTESIAN_POINT('Ctrl Pts',(51.0191714801764,-36.8060871110687,
40.0889901646429));
#168204=CARTESIAN_POINT('Ctrl Pts',(51.01512897876,-36.8283529098803,40.1045963098259));
#168205=CARTESIAN_POINT('Ctrl Pts',(51.008609334901,-36.8513189052339,40.1176634650745));
#168206=CARTESIAN_POINT('Ctrl Pts',(51.0056832284514,-36.8616263619877,
40.1235281853075));
#168207=CARTESIAN_POINT('Ctrl Pts',(51.0022583633859,-36.8720751481068,
40.1288820140926));
#168208=CARTESIAN_POINT('Ctrl Pts',(50.9983419378324,-36.8825875141943,
40.1336621774101));
#168209=CARTESIAN_POINT('Ctrl Pts',(50.9966399122601,-36.8871560463067,
40.1357395717319));
#168210=CARTESIAN_POINT('Ctrl Pts',(50.9948449951612,-36.8917363891938,
40.1377083672884));
#168211=CARTESIAN_POINT('Ctrl Pts',(50.9929577488698,-36.8963220336349,
40.1395632548792));
#168212=CARTESIAN_POINT('Ctrl Pts',(50.98635238685,-36.9123717891788,40.146055361447));
#168213=CARTESIAN_POINT('Ctrl Pts',(50.9786159896081,-36.9284864868682,
40.151152097463));
#168214=CARTESIAN_POINT('Ctrl Pts',(50.9697726815835,-36.9443870542876,
40.1546258197409));
#168215=CARTESIAN_POINT('Ctrl Pts',(50.9653510275712,-36.9523373379973,
40.1563626808798));
#168216=CARTESIAN_POINT('Ctrl Pts',(50.9606526463565,-36.960234089495,40.1576937882008));
#168217=CARTESIAN_POINT('Ctrl Pts',(50.9556805599063,-36.968042429379,40.1585906813668));
#168218=CARTESIAN_POINT('Ctrl Pts',(50.9531945166812,-36.9719465993211,
40.1590391279498));
#168219=CARTESIAN_POINT('Ctrl Pts',(50.9506400472468,-36.9758286664321,
40.1593790209175));
#168220=CARTESIAN_POINT('Ctrl Pts',(50.948017529914,-36.9796842711995,40.1596068022931));
#168221=CARTESIAN_POINT('Ctrl Pts',(50.9453950125812,-36.9835398759669,
40.1598345836687));
#168222=CARTESIAN_POINT('Ctrl Pts',(50.9427044459693,-36.987369017388,40.1599502506864));
#168223=CARTESIAN_POINT('Ctrl Pts',(50.9399462128201,-36.9911673391708,
40.1599502534424));
#168224=CARTESIAN_POINT('',(50.9219998155899,-37.015868435856,40.1599502534424));
#168225=CARTESIAN_POINT('Origin',(5.52946850001198E-15,5.78623384841323E-15,
40.1599502534424));
#168226=CARTESIAN_POINT('',(50.5905785208484,-37.1493329797261,39.8576902534424));
#168227=CARTESIAN_POINT('Ctrl Pts',(50.9219998155899,-37.015868435856,40.1599502534424));
#168228=CARTESIAN_POINT('Ctrl Pts',(50.919752770815,-37.0189596418149,40.1599502447858));
#168229=CARTESIAN_POINT('Ctrl Pts',(50.9174732734523,-37.0220143142659,
40.1598744685927));
#168230=CARTESIAN_POINT('Ctrl Pts',(50.9151633654183,-37.0250315520725,
40.1597246934279));
#168231=CARTESIAN_POINT('Ctrl Pts',(50.9018149465639,-37.0424674644257,
40.1588591777435));
#168232=CARTESIAN_POINT('Ctrl Pts',(50.8874508031645,-37.0586566148276,
40.1555254706022));
#168233=CARTESIAN_POINT('Ctrl Pts',(50.8724683783922,-37.0734189189002,
40.1500631826386));
#168234=CARTESIAN_POINT('Ctrl Pts',(50.8664256218263,-37.0793728957243,
40.1478601162485));
#168235=CARTESIAN_POINT('Ctrl Pts',(50.8602822855873,-37.085095235135,40.1453112228309));
#168236=CARTESIAN_POINT('Ctrl Pts',(50.8540642095546,-37.0905759575255,
40.1424401896328));
#168237=CARTESIAN_POINT('Ctrl Pts',(50.851770117014,-37.0925980113388,40.1413809526905));
#168238=CARTESIAN_POINT('Ctrl Pts',(50.8494658679866,-37.0945870443967,
40.1402777640511));
#168239=CARTESIAN_POINT('Ctrl Pts',(50.8471527697479,-37.0965424902852,
40.1391317641987));
#168240=CARTESIAN_POINT('Ctrl Pts',(50.8428157105503,-37.1002089513262,
40.1369830144753));
#168241=CARTESIAN_POINT('Ctrl Pts',(50.8384475408394,-37.1037573324717,
40.1346837565849));
#168242=CARTESIAN_POINT('Ctrl Pts',(50.8340568779947,-37.1071839000978,
40.1322415082996));
#168243=CARTESIAN_POINT('Ctrl Pts',(50.8186895580382,-37.119176886789,40.1236936393008));
#168244=CARTESIAN_POINT('Ctrl Pts',(50.803046693569,-37.12967765523,40.113394140767));
#168245=CARTESIAN_POINT('Ctrl Pts',(50.7874977752343,-37.1385261411558,
40.101665321223));
#168246=CARTESIAN_POINT('Ctrl Pts',(50.7797233160669,-37.1429503841186,
40.095800911451));
#168247=CARTESIAN_POINT('Ctrl Pts',(50.7719723442506,-37.1469615570463,
40.0895791707949));
#168248=CARTESIAN_POINT('Ctrl Pts',(50.7642910532777,-37.1505396571686,
40.0830403822906));
#168249=CARTESIAN_POINT('Ctrl Pts',(50.7604504077912,-37.1523287072298,
40.0797709880385));
#168250=CARTESIAN_POINT('Ctrl Pts',(50.75662718261,-37.1540094891595,40.0764223317514));
#168251=CARTESIAN_POINT('Ctrl Pts',(50.7528271523479,-37.1555795029286,
40.0729994484778));
#168252=CARTESIAN_POINT('Ctrl Pts',(50.7490271220858,-37.1571495166978,
40.0695765652042));
#168253=CARTESIAN_POINT('Ctrl Pts',(50.7452503160124,-37.1586086360831,
40.0660793733488));
#168254=CARTESIAN_POINT('Ctrl Pts',(50.7415024502312,-37.1599546198238,
40.0625130768817));
#168255=CARTESIAN_POINT('Ctrl Pts',(50.7414704887854,-37.1599660982462,
40.0624826638418));
#168256=CARTESIAN_POINT('Ctrl Pts',(50.7414385295747,-37.1599775684899,
40.0624522459912));
#168257=CARTESIAN_POINT('Ctrl Pts',(50.7414065726022,-37.159989030554,40.0624218233329));
#168258=CARTESIAN_POINT('Ctrl Pts',(50.7250856801828,-37.1658428740577,
40.0468845275901));
#168259=CARTESIAN_POINT('Ctrl Pts',(50.709357947548,-37.1696950534575,40.0302263329242));
#168260=CARTESIAN_POINT('Ctrl Pts',(50.6943448053384,-37.1717050161488,
40.012751588475));
#168261=CARTESIAN_POINT('Ctrl Pts',(50.6788239286281,-37.1737829544436,
39.994685859772));
#168262=CARTESIAN_POINT('Ctrl Pts',(50.6640659431905,-37.1738916781074,
39.9757460620494));
#168263=CARTESIAN_POINT('Ctrl Pts',(50.6502224036994,-37.1721581240049,
39.9562444559131));
#168264=CARTESIAN_POINT('Ctrl Pts',(50.636642197459,-37.1704575457491,39.9371138113609));
#168265=CARTESIAN_POINT('Ctrl Pts',(50.6239412983375,-37.1669834785894,
39.9174410654346));
#168266=CARTESIAN_POINT('Ctrl Pts',(50.6122904324844,-37.161816682268,39.8975196504132));
#168267=CARTESIAN_POINT('Ctrl Pts',(50.6045721423186,-37.1583938608452,
39.8843224113766));
#168268=CARTESIAN_POINT('Ctrl Pts',(50.5973152449644,-37.154227389024,39.8710160447127));
#168269=CARTESIAN_POINT('Ctrl Pts',(50.5905785208484,-37.1493329797261,
39.8576902534424));
#168270=CARTESIAN_POINT('',(50.3023253561995,-36.9399086546487,39.2875012672119));
#168271=CARTESIAN_POINT('',(50.5905785208484,-37.1493329797261,39.8576902534424));
#168272=CARTESIAN_POINT('',(46.5911245387429,-41.5228599914563,39.2875012672119));
#168273=CARTESIAN_POINT('Origin',(5.53234440788222E-15,0.,39.2875012672119));
#168274=CARTESIAN_POINT('',(46.8559036426985,-41.7612723673363,39.8576902534424));
#168275=CARTESIAN_POINT('',(46.5911245387429,-41.5228599914563,39.2875012672119));
#168276=CARTESIAN_POINT('',(46.7942619810916,-42.1132001506002,40.1599502534424));
#168277=CARTESIAN_POINT('Ctrl Pts',(46.8559036426985,-41.7612723673363,
39.8576902534424));
#168278=CARTESIAN_POINT('Ctrl Pts',(46.8650486462049,-41.7695067430954,
39.877383612036));
#168279=CARTESIAN_POINT('Ctrl Pts',(46.8728586744677,-41.7791634256542,
39.8969946442124));
#168280=CARTESIAN_POINT('Ctrl Pts',(46.8792591175167,-41.7900688448319,
39.9162525288229));
#168281=CARTESIAN_POINT('Ctrl Pts',(46.8857881704163,-41.8011933963915,
39.9358973794046));
#168282=CARTESIAN_POINT('Ctrl Pts',(46.8908511403511,-41.8136179609666,
39.9551762199718));
#168283=CARTESIAN_POINT('Ctrl Pts',(46.8943401533967,-41.8272034165397,
39.9738152034217));
#168284=CARTESIAN_POINT('Ctrl Pts',(46.8976936214484,-41.8402610894794,
39.9917300792612));
#168285=CARTESIAN_POINT('Ctrl Pts',(46.8995933993941,-41.8543920170376,
40.0090551158084));
#168286=CARTESIAN_POINT('Ctrl Pts',(46.8999101480297,-41.8695030436287,
40.0255394551492));
#168287=CARTESIAN_POINT('Ctrl Pts',(46.9001534633402,-41.8811108098924,
40.0382021526122));
#168288=CARTESIAN_POINT('Ctrl Pts',(46.8994620807995,-41.8932975750523,
40.050368778211));
#168289=CARTESIAN_POINT('Ctrl Pts',(46.8977610424072,-41.9060298852855,
40.0619155352442));
#168290=CARTESIAN_POINT('Ctrl Pts',(46.8977565842889,-41.9060632544,40.0619457972351));
#168291=CARTESIAN_POINT('Ctrl Pts',(46.8977521185701,-41.90609662777,40.0619760547305));
#168292=CARTESIAN_POINT('Ctrl Pts',(46.8977476452508,-41.9061300053924,
40.0620063077269));
#168293=CARTESIAN_POINT('Ctrl Pts',(46.8972680144604,-41.9097087652732,
40.06525004417));
#168294=CARTESIAN_POINT('Ctrl Pts',(46.8967002823076,-41.9133346546842,
40.0684393223556));
#168295=CARTESIAN_POINT('Ctrl Pts',(46.8960451360319,-41.9170027866176,
40.0715697951759));
#168296=CARTESIAN_POINT('Ctrl Pts',(46.8923993959694,-41.9374151067973,
40.0889901646393));
#168297=CARTESIAN_POINT('Ctrl Pts',(46.8860516300673,-41.9591363747677,
40.1045963098194));
#168298=CARTESIAN_POINT('Ctrl Pts',(46.8771671013008,-41.9812950716373,
40.1176634650663));
#168299=CARTESIAN_POINT('Ctrl Pts',(46.8731796017524,-41.9912402016585,
40.1235281853025));
#168300=CARTESIAN_POINT('Ctrl Pts',(46.8686813028982,-42.0012737523564,
40.1288820140903));
#168301=CARTESIAN_POINT('Ctrl Pts',(46.863687490459,-42.0113191526625,40.1336621774101));
#168302=CARTESIAN_POINT('Ctrl Pts',(46.8615172471197,-42.0156847477605,
40.1357395717319));
#168303=CARTESIAN_POINT('Ctrl Pts',(46.8592533865613,-42.020052379124,40.1377083672883));
#168304=CARTESIAN_POINT('Ctrl Pts',(46.8568971484361,-42.0244156319704,
40.1395632548791));
#168305=CARTESIAN_POINT('Ctrl Pts',(46.8486503149976,-42.0396870169328,
40.1460553614469));
#168306=CARTESIAN_POINT('Ctrl Pts',(46.8392718539638,-42.0549047629073,
40.1511520974629));
#168307=CARTESIAN_POINT('Ctrl Pts',(46.8288149286284,-42.0697938479567,
40.1546258197408));
#168308=CARTESIAN_POINT('Ctrl Pts',(46.8235864659607,-42.0772383904814,
40.1563626808798));
#168309=CARTESIAN_POINT('Ctrl Pts',(46.8180883876711,-42.0846007681799,
40.1576937882008));
#168310=CARTESIAN_POINT('Ctrl Pts',(46.8123273450619,-42.0918466086052,
40.1585906813668));
#168311=CARTESIAN_POINT('Ctrl Pts',(46.8094468237573,-42.0954695288179,
40.1590391279498));
#168312=CARTESIAN_POINT('Ctrl Pts',(46.8065005614644,-42.0990633147947,
40.1593790209175));
#168313=CARTESIAN_POINT('Ctrl Pts',(46.8034893901146,-42.102623670449,40.1596068022931));
#168314=CARTESIAN_POINT('Ctrl Pts',(46.8004782187648,-42.1061840261034,
40.1598345836687));
#168315=CARTESIAN_POINT('Ctrl Pts',(46.79740213709,-42.1097109502939,40.1599502506865));
#168316=CARTESIAN_POINT('Ctrl Pts',(46.7942619810916,-42.1132001506002,
40.1599502534424));
#168317=CARTESIAN_POINT('',(46.7738319284257,-42.1358900227696,40.1599502534424));
#168318=CARTESIAN_POINT('Origin',(5.53970586838553E-15,5.79887594550813E-15,
40.1599502534424));
#168319=CARTESIAN_POINT('',(46.4302753505424,-42.2339804752702,39.8576902534424));
#168320=CARTESIAN_POINT('Ctrl Pts',(46.7738319284257,-42.1358900227696,
40.1599502534424));
#168321=CARTESIAN_POINT('Ctrl Pts',(46.7712740741886,-42.1387294146415,
40.1599502447857));
#168322=CARTESIAN_POINT('Ctrl Pts',(46.7686877639338,-42.1415290809209,
40.1598744685927));
#168323=CARTESIAN_POINT('Ctrl Pts',(46.7660751225865,-42.144288338846,40.1597246934279));
#168324=CARTESIAN_POINT('Ctrl Pts',(46.7509772786445,-42.1602334457358,
40.1588591777436));
#168325=CARTESIAN_POINT('Ctrl Pts',(46.7349995965139,-42.1748324484412,
40.1555254706028));
#168326=CARTESIAN_POINT('Ctrl Pts',(46.7185561660745,-42.1879477932292,
40.1500631826399));
#168327=CARTESIAN_POINT('Ctrl Pts',(46.7119241523123,-42.1932375134886,
40.1478601162495));
#168328=CARTESIAN_POINT('Ctrl Pts',(46.7052163225658,-42.1982863518299,
40.1453112228315));
#168329=CARTESIAN_POINT('Ctrl Pts',(46.6984594183138,-42.2030870843185,
40.1424401896328));
#168330=CARTESIAN_POINT('Ctrl Pts',(46.6959665308745,-42.2048582631416,
40.1413809526906));
#168331=CARTESIAN_POINT('Ctrl Pts',(46.6934669941954,-42.2065955404584,
40.1402777640511));
#168332=CARTESIAN_POINT('Ctrl Pts',(46.6909621675971,-42.2082984896054,
40.1391317641987));
#168333=CARTESIAN_POINT('Ctrl Pts',(46.6862656177254,-42.2114915192562,
40.1369830144753));
#168334=CARTESIAN_POINT('Ctrl Pts',(46.6815504704771,-42.2145638639314,
40.134683756585));
#168335=CARTESIAN_POINT('Ctrl Pts',(46.6768256862946,-42.2175127112216,
40.1322415082996));
#168336=CARTESIAN_POINT('Ctrl Pts',(46.6602889416559,-42.2278336767372,
40.1236936393009));
#168337=CARTESIAN_POINT('Ctrl Pts',(46.6436341412467,-42.236641796286,40.113394140767));
#168338=CARTESIAN_POINT('Ctrl Pts',(46.6272454828774,-42.243816504741,40.101665321223));
#168339=CARTESIAN_POINT('Ctrl Pts',(46.6190511536928,-42.2474038589685,
40.095800911451));
#168340=CARTESIAN_POINT('Ctrl Pts',(46.610923360769,-42.2505828610984,40.0895791707949));
#168341=CARTESIAN_POINT('Ctrl Pts',(46.6029101354046,-42.2533384464725,
40.0830403822906));
#168342=CARTESIAN_POINT('Ctrl Pts',(46.5989035227223,-42.2547162391596,
40.0797709880385));
#168343=CARTESIAN_POINT('Ctrl Pts',(46.5949255520165,-42.2559881777371,
40.0764223317514));
#168344=CARTESIAN_POINT('Ctrl Pts',(46.5909822275911,-42.2571523794829,
40.0729994484778));
#168345=CARTESIAN_POINT('Ctrl Pts',(46.5870389031658,-42.2583165812286,
40.0695765652042));
#168346=CARTESIAN_POINT('Ctrl Pts',(46.5831302673242,-42.2593729236704,
40.0660793733488));
#168347=CARTESIAN_POINT('Ctrl Pts',(46.5792622391319,-42.2603197753207,
40.0625130768817));
#168348=CARTESIAN_POINT('Ctrl Pts',(46.5792292529523,-42.2603278499823,
40.0624826638418));
#168349=CARTESIAN_POINT('Ctrl Pts',(46.5791962698506,-42.2603359167436,
40.0624522459912));
#168350=CARTESIAN_POINT('Ctrl Pts',(46.5791632898298,-42.2603439756041,
40.0624218233329));
#168351=CARTESIAN_POINT('Ctrl Pts',(46.5623199117009,-42.264459753337,40.0468845275898));
#168352=CARTESIAN_POINT('Ctrl Pts',(46.5462756748379,-42.2666468343719,
40.0302263329236));
#168353=CARTESIAN_POINT('Ctrl Pts',(46.5311346778806,-42.2670764855932,
40.0127515884741));
#168354=CARTESIAN_POINT('Ctrl Pts',(46.51548162246,-42.2675206673335,39.9946858597709));
#168355=CARTESIAN_POINT('Ctrl Pts',(46.5007931180932,-42.2660861658588,
39.975746062048));
#168356=CARTESIAN_POINT('Ctrl Pts',(46.4872066207061,-42.2629150644377,
39.9562444559114));
#168357=CARTESIAN_POINT('Ctrl Pts',(46.4738785670881,-42.2598042840382,
39.9371138113589));
#168358=CARTESIAN_POINT('Ctrl Pts',(46.4616103837223,-42.2550216427145,
39.9174410654322));
#168359=CARTESIAN_POINT('Ctrl Pts',(46.4505634198108,-42.2486653035403,
39.8975196504106));
#168360=CARTESIAN_POINT('Ctrl Pts',(46.44324519351,-42.2444544516815,39.8843224113748));
#168361=CARTESIAN_POINT('Ctrl Pts',(46.436463565096,-42.2395522519007,39.8710160447118));
#168362=CARTESIAN_POINT('Ctrl Pts',(46.4302753505424,-42.2339804752702,
39.8576902534424));
#168363=CARTESIAN_POINT('',(46.1654920697611,-41.9955727382252,39.2875012672119));
#168364=CARTESIAN_POINT('',(46.4302753505424,-42.2339804752702,39.8576902534424));
#168365=CARTESIAN_POINT('',(41.995572738225,-46.1654920697613,39.2875012672119));
#168366=CARTESIAN_POINT('Origin',(5.53234440788222E-15,0.,39.2875012672119));
#168367=CARTESIAN_POINT('',(42.23398047527,-46.4302753505426,39.8576902534424));
#168368=CARTESIAN_POINT('',(41.995572738225,-46.1654920697613,39.2875012672119));
#168369=CARTESIAN_POINT('',(42.1358900227694,-46.7738319284258,40.1599502534424));
#168370=CARTESIAN_POINT('Ctrl Pts',(42.23398047527,-46.4302753505426,39.8576902534424));
#168371=CARTESIAN_POINT('Ctrl Pts',(42.2422146548454,-46.439420530692,39.8773836120339));
#168372=CARTESIAN_POINT('Ctrl Pts',(42.2489725007673,-46.4498406831845,
39.8969946442083));
#168373=CARTESIAN_POINT('Ctrl Pts',(42.2541979548115,-46.4613553898097,
39.9162525288168));
#168374=CARTESIAN_POINT('Ctrl Pts',(42.2595284085967,-46.4731014717765,
39.9358973793964));
#168375=CARTESIAN_POINT('Ctrl Pts',(42.2632649224108,-46.4859871977518,
39.9551762199615));
#168376=CARTESIAN_POINT('Ctrl Pts',(42.2653147554845,-46.4998629319477,
39.9738152034094));
#168377=CARTESIAN_POINT('Ctrl Pts',(42.2672849544016,-46.5131996064485,
39.9917300792466));
#168378=CARTESIAN_POINT('Ctrl Pts',(42.2676972410237,-46.5274517041735,
40.0090551157917));
#168379=CARTESIAN_POINT('Ctrl Pts',(42.2664327220907,-46.5425130602251,
40.0255394551308));
#168380=CARTESIAN_POINT('Ctrl Pts',(42.2654613625255,-46.5540826713113,
40.0382021526004));
#168381=CARTESIAN_POINT('Ctrl Pts',(42.2634999036159,-46.5661304069476,
40.0503687782054));
#168382=CARTESIAN_POINT('Ctrl Pts',(42.2604772948659,-46.5786151613301,
40.0619155352442));
#168383=CARTESIAN_POINT('Ctrl Pts',(42.2604693731474,-46.5786478816448,
40.0619457972351));
#168384=CARTESIAN_POINT('Ctrl Pts',(42.2604614434252,-46.5786806053973,
40.0619760547304));
#168385=CARTESIAN_POINT('Ctrl Pts',(42.2604535056997,-46.5787133325844,
40.0620063077269));
#168386=CARTESIAN_POINT('Ctrl Pts',(42.2596024201061,-46.5822223525746,
40.06525004417));
#168387=CARTESIAN_POINT('Ctrl Pts',(42.2586587894014,-46.5857690348146,
40.0684393223556));
#168388=CARTESIAN_POINT('Ctrl Pts',(42.2576238078915,-46.5893485909041,
40.0715697951759));
#168389=CARTESIAN_POINT('Ctrl Pts',(42.2518643711122,-46.6092680066592,
40.0889901646458));
#168390=CARTESIAN_POINT('Ctrl Pts',(42.2432808881705,-46.6302067610441,
40.1045963098309));
#168391=CARTESIAN_POINT('Ctrl Pts',(42.2321288152444,-46.6513153841229,
40.1176634650808));
#168392=CARTESIAN_POINT('Ctrl Pts',(42.2271236104809,-46.6607892264734,
40.1235281853113));
#168393=CARTESIAN_POINT('Ctrl Pts',(42.2216011621471,-46.6702976120563,
40.1288820140942));
#168394=CARTESIAN_POINT('Ctrl Pts',(42.2155846760829,-46.6797659870606,
40.13366217741));
#168395=CARTESIAN_POINT('Ctrl Pts',(42.2129699926169,-46.6838808147706,
40.1357395717318));
#168396=CARTESIAN_POINT('Ctrl Pts',(42.210261991929,-46.6879878819273,40.1377083672883));
#168397=CARTESIAN_POINT('Ctrl Pts',(42.2074625774079,-46.6920809384678,
40.1395632548791));
#168398=CARTESIAN_POINT('Ctrl Pts',(42.1976646265838,-46.7064066363594,
40.1460553614469));
#168399=CARTESIAN_POINT('Ctrl Pts',(42.1867468541397,-46.7205607018095,
40.1511520974629));
#168400=CARTESIAN_POINT('Ctrl Pts',(42.1747908797557,-46.7342751765573,
40.1546258197408));
#168401=CARTESIAN_POINT('Ctrl Pts',(42.1688128925637,-46.7411324139312,
40.1563626808798));
#168402=CARTESIAN_POINT('Ctrl Pts',(42.1625753552954,-46.7478797540798,
40.1576937882008));
#168403=CARTESIAN_POINT('Ctrl Pts',(42.1560884757157,-46.7544837081024,
40.1585906813668));
#168404=CARTESIAN_POINT('Ctrl Pts',(42.1528450359258,-46.7577856851136,
40.1590391279498));
#168405=CARTESIAN_POINT('Ctrl Pts',(42.1495392606406,-46.761051815685,40.1593790209175));
#168406=CARTESIAN_POINT('Ctrl Pts',(42.1461724262973,-46.7642779142247,
40.1596068022931));
#168407=CARTESIAN_POINT('Ctrl Pts',(42.142805591954,-46.7675040127644,40.1598345836687));
#168408=CARTESIAN_POINT('Ctrl Pts',(42.1393776974107,-46.7706900780048,
40.1599502506864));
#168409=CARTESIAN_POINT('Ctrl Pts',(42.1358900227694,-46.7738319284258,
40.1599502534424));
#168410=CARTESIAN_POINT('',(42.1132001506,-46.7942619810918,40.1599502534424));
#168411=CARTESIAN_POINT('Origin',(5.55120861436579E-15,5.81037869148839E-15,
40.1599502534424));
#168412=CARTESIAN_POINT('',(41.7612723673362,-46.8559036426986,39.8576902534424));
#168413=CARTESIAN_POINT('Ctrl Pts',(42.1132001506,-46.7942619810918,40.1599502534424));
#168414=CARTESIAN_POINT('Ctrl Pts',(42.1103595112871,-46.7968184499053,
40.1599502447858));
#168415=CARTESIAN_POINT('Ctrl Pts',(42.1074947242967,-46.7993324362834,
40.1598744685927));
#168416=CARTESIAN_POINT('Ctrl Pts',(42.1046079742813,-46.8018034833197,
40.1597246934279));
#168417=CARTESIAN_POINT('Ctrl Pts',(42.0879261203911,-46.8160830868174,
40.1588591777437));
#168418=CARTESIAN_POINT('Ctrl Pts',(42.0705099543599,-46.8289319920969,
40.1555254706039));
#168419=CARTESIAN_POINT('Ctrl Pts',(42.0527856759201,-46.8402566831377,
40.1500631826426));
#168420=CARTESIAN_POINT('Ctrl Pts',(42.0456370666904,-46.8448241915513,
40.1478601162516));
#168421=CARTESIAN_POINT('Ctrl Pts',(42.0384382358211,-46.8491442126946,
40.1453112228326));
#168422=CARTESIAN_POINT('Ctrl Pts',(42.031216533405,-46.853212357452,40.1424401896328));
#168423=CARTESIAN_POINT('Ctrl Pts',(42.0285521636633,-46.854713255879,40.1413809526905));
#168424=CARTESIAN_POINT('Ctrl Pts',(42.0258847247795,-46.856179743481,40.1402777640511));
#168425=CARTESIAN_POINT('Ctrl Pts',(42.0232156132261,-46.8576115380194,
40.1391317641987));
#168426=CARTESIAN_POINT('Ctrl Pts',(42.0182110290634,-46.8602961527789,
40.1369830144753));
#168427=CARTESIAN_POINT('Ctrl Pts',(42.0132005644175,-46.8628587997325,
40.1346837565849));
#168428=CARTESIAN_POINT('Ctrl Pts',(42.0081934246215,-46.8652976184988,
40.1322415082996));
#168429=CARTESIAN_POINT('Ctrl Pts',(41.9906684353354,-46.8738334841809,
40.1236936393008));
#168430=CARTESIAN_POINT('Ctrl Pts',(41.9731841724648,-46.8808524512363,
40.113394140767));
#168431=CARTESIAN_POINT('Ctrl Pts',(41.9561353316316,-46.8862747746134,
40.101665321223));
#168432=CARTESIAN_POINT('Ctrl Pts',(41.9476109112151,-46.8889859363019,
40.095800911451));
#168433=CARTESIAN_POINT('Ctrl Pts',(41.939195346984,-46.8912979378214,40.0895791707949));
#168434=CARTESIAN_POINT('Ctrl Pts',(41.930937981802,-46.8932008176774,40.0830403822906));
#168435=CARTESIAN_POINT('Ctrl Pts',(41.926809299211,-46.8941522576054,40.0797709880385));
#168436=CARTESIAN_POINT('Ctrl Pts',(41.92272016646,-46.8950014172055,40.0764223317514));
#168437=CARTESIAN_POINT('Ctrl Pts',(41.918676751759,-46.8957470516899,40.0729994484778));
#168438=CARTESIAN_POINT('Ctrl Pts',(41.9146333370581,-46.8964926861744,
40.0695765652042));
#168439=CARTESIAN_POINT('Ctrl Pts',(41.9106356952805,-46.8971346781637,
40.0660793733488));
#168440=CARTESIAN_POINT('Ctrl Pts',(41.9066898836034,-46.8976720238188,
40.0625130768816));
#168441=CARTESIAN_POINT('Ctrl Pts',(41.9066562340936,-46.8976766062519,
40.0624826638418));
#168442=CARTESIAN_POINT('Ctrl Pts',(41.9066225884706,-46.8976811811497,
40.0624522459912));
#168443=CARTESIAN_POINT('Ctrl Pts',(41.9065889467375,-46.897685748512,40.0624218233329));
#168444=CARTESIAN_POINT('Ctrl Pts',(41.889407622474,-46.9000183671518,40.0468845275891));
#168445=CARTESIAN_POINT('Ctrl Pts',(41.873222665399,-46.9005163877045,40.0302263329222));
#168446=CARTESIAN_POINT('Ctrl Pts',(41.8581197016247,-46.899361020107,40.012751588472));
#168447=CARTESIAN_POINT('Ctrl Pts',(41.8425059656445,-46.8981665787446,
39.9946858597683));
#168448=CARTESIAN_POINT('Ctrl Pts',(41.8280478726759,-46.8952045688299,
39.9757460620449));
#168449=CARTESIAN_POINT('Ctrl Pts',(41.8148672739013,-46.8906306633408,
39.9562444559078));
#168450=CARTESIAN_POINT('Ctrl Pts',(41.8019373978504,-46.8861437631587,
39.9371138113554));
#168451=CARTESIAN_POINT('Ctrl Pts',(41.7902363430249,-46.8801049472901,
39.9174410654289));
#168452=CARTESIAN_POINT('Ctrl Pts',(41.7799143139038,-46.8726287066454,
39.8975196504074));
#168453=CARTESIAN_POINT('Ctrl Pts',(41.773076331487,-46.8676759593248,39.8843224113726));
#168454=CARTESIAN_POINT('Ctrl Pts',(41.7668442729534,-46.8620917411111,
39.8710160447107));
#168455=CARTESIAN_POINT('Ctrl Pts',(41.7612723673362,-46.8559036426986,
39.8576902534424));
#168456=CARTESIAN_POINT('',(41.5228599914562,-46.5911245387431,39.2875012672119));
#168457=CARTESIAN_POINT('',(41.7612723673362,-46.8559036426986,39.8576902534424));
#168458=CARTESIAN_POINT('',(36.9399086546485,-50.3023253561996,39.2875012672119));
#168459=CARTESIAN_POINT('Origin',(5.53234440788222E-15,0.,39.2875012672119));
#168460=CARTESIAN_POINT('',(37.149332979726,-50.5905785208485,39.8576902534424));
#168461=CARTESIAN_POINT('',(36.9399086546485,-50.3023253561996,39.2875012672119));
#168462=CARTESIAN_POINT('',(37.0158684358559,-50.9219998155901,40.1599502534424));
#168463=CARTESIAN_POINT('Ctrl Pts',(37.149332979726,-50.5905785208485,39.8576902534424));
#168464=CARTESIAN_POINT('Ctrl Pts',(37.156566119978,-50.6005343088827,39.8773836120369));
#168465=CARTESIAN_POINT('Ctrl Pts',(37.1621977431866,-50.6116037659405,
39.8969946442141));
#168466=CARTESIAN_POINT('Ctrl Pts',(37.1661909570584,-50.6236016024811,
39.9162525288254));
#168467=CARTESIAN_POINT('Ctrl Pts',(37.1702644101629,-50.6358405223268,
39.9358973794081));
#168468=CARTESIAN_POINT('Ctrl Pts',(37.1726335298287,-50.6490462309966,
39.9551762199761));
#168469=CARTESIAN_POINT('Ctrl Pts',(37.1732217245291,-50.6630602183728,
39.9738152034268));
#168470=CARTESIAN_POINT('Ctrl Pts',(37.1737870683986,-50.6765297750435,
39.9917300792672));
#168471=CARTESIAN_POINT('Ctrl Pts',(37.1727073465962,-50.6907468939765,
40.0090551158152));
#168472=CARTESIAN_POINT('Ctrl Pts',(37.1698754144249,-50.7055935641267,
40.0255394551566));
#168473=CARTESIAN_POINT('Ctrl Pts',(37.1677000224016,-50.716998260943,40.038202152617));
#168474=CARTESIAN_POINT('Ctrl Pts',(37.1644899772785,-50.7287749695296,
40.0503687782133));
#168475=CARTESIAN_POINT('Ctrl Pts',(37.1601789145086,-50.7408753824653,
40.0619155352442));
#168476=CARTESIAN_POINT('Ctrl Pts',(37.160167615982,-50.7409070954897,40.0619457972351));
#168477=CARTESIAN_POINT('Ctrl Pts',(37.160156309136,-50.7409388110964,40.0619760547305));
#168478=CARTESIAN_POINT('Ctrl Pts',(37.1601449939716,-50.7409705292822,
40.0620063077269));
#168479=CARTESIAN_POINT('Ctrl Pts',(37.1589317782469,-50.7443713638246,
40.06525004417));
#168480=CARTESIAN_POINT('Ctrl Pts',(37.1576225876056,-50.7477999807007,
40.0684393223556));
#168481=CARTESIAN_POINT('Ctrl Pts',(37.1562191103355,-50.7512517425806,
40.0715697951759));
#168482=CARTESIAN_POINT('Ctrl Pts',(37.1484090784384,-50.7704600126088,
40.088990164639));
#168483=CARTESIAN_POINT('Ctrl Pts',(37.1376839209011,-50.7903868440169,
40.1045963098188));
#168484=CARTESIAN_POINT('Ctrl Pts',(37.1243864882723,-50.8102141227971,
40.1176634650657));
#168485=CARTESIAN_POINT('Ctrl Pts',(37.1184184163579,-50.8191128800934,
40.1235281853021));
#168486=CARTESIAN_POINT('Ctrl Pts',(37.1119323236356,-50.8279919247151,
40.1288820140901));
#168487=CARTESIAN_POINT('Ctrl Pts',(37.1049590818167,-50.8367795369354,
40.1336621774101));
#168488=CARTESIAN_POINT('Ctrl Pts',(37.1019286052431,-50.8405985143441,
40.1357395717319));
#168489=CARTESIAN_POINT('Ctrl Pts',(37.0988061338479,-50.8444000194068,
40.1377083672883));
#168490=CARTESIAN_POINT('Ctrl Pts',(37.0955942139022,-50.8481780352573,
40.1395632548791));
#168491=CARTESIAN_POINT('Ctrl Pts',(37.0843524940921,-50.8614010907341,
40.146055361447));
#168492=CARTESIAN_POINT('Ctrl Pts',(37.0720150276373,-50.8743364007568,
40.1511520974629));
#168493=CARTESIAN_POINT('Ctrl Pts',(37.058690996362,-50.8867260065478,40.1546258197408));
#168494=CARTESIAN_POINT('Ctrl Pts',(37.0520289807244,-50.8929208094433,
40.1563626808798));
#168495=CARTESIAN_POINT('Ctrl Pts',(37.045120324241,-50.8989791867713,40.1576937882008));
#168496=CARTESIAN_POINT('Ctrl Pts',(37.0379786793009,-50.9048689000888,
40.1585906813668));
#168497=CARTESIAN_POINT('Ctrl Pts',(37.0344078568308,-50.9078137567476,
40.1590391279498));
#168498=CARTESIAN_POINT('Ctrl Pts',(37.030778787319,-50.9107164475034,40.1593790209175));
#168499=CARTESIAN_POINT('Ctrl Pts',(37.0270931777238,-50.9135729431178,
40.1596068022931));
#168500=CARTESIAN_POINT('Ctrl Pts',(37.0234075681286,-50.9164294387322,
40.1598345836687));
#168501=CARTESIAN_POINT('Ctrl Pts',(37.019665417447,-50.9192397378251,40.1599502506865));
#168502=CARTESIAN_POINT('Ctrl Pts',(37.0158684358559,-50.92199981559,40.1599502534424));
#168503=CARTESIAN_POINT('',(36.9911673391707,-50.9399462128202,40.1599502534424));
#168504=CARTESIAN_POINT('Origin',(5.56385071146069E-15,5.82061605986194E-15,
40.1599502534424));
#168505=CARTESIAN_POINT('',(36.6347241449654,-50.9644637245894,39.8576902534424));
#168506=CARTESIAN_POINT('Ctrl Pts',(36.9911673391707,-50.9399462128202,
40.1599502534424));
#168507=CARTESIAN_POINT('Ctrl Pts',(36.9880750374206,-50.942191749368,40.1599502447858));
#168508=CARTESIAN_POINT('Ctrl Pts',(36.9849631609003,-50.944392512084,40.1598744685927));
#168509=CARTESIAN_POINT('Ctrl Pts',(36.9818339300542,-50.9465482749232,
40.1597246934279));
#168510=CARTESIAN_POINT('Ctrl Pts',(36.9637508360892,-50.9590059247115,
40.1588591777434));
#168511=CARTESIAN_POINT('Ctrl Pts',(36.9450870013077,-50.9699639572754,
40.1555254706016));
#168512=CARTESIAN_POINT('Ctrl Pts',(36.9262760657617,-50.9793739188881,
40.150063182637));
#168513=CARTESIAN_POINT('Ctrl Pts',(36.9186891827323,-50.9831691728718,
40.1478601162473));
#168514=CARTESIAN_POINT('Ctrl Pts',(36.9110782226468,-50.9867130457559,
40.1453112228302));
#168515=CARTESIAN_POINT('Ctrl Pts',(36.9034708445588,-50.9900040313322,
40.1424401896328));
#168516=CARTESIAN_POINT('Ctrl Pts',(36.9006641839072,-50.9912182052059,
40.1413809526905));
#168517=CARTESIAN_POINT('Ctrl Pts',(36.8978580678373,-50.9923978359479,
40.1402777640511));
#168518=CARTESIAN_POINT('Ctrl Pts',(36.8950539146734,-50.9935427888371,
40.1391317641987));
#168519=CARTESIAN_POINT('Ctrl Pts',(36.8897961274911,-50.9956895755043,
40.1369830144753));
#168520=CARTESIAN_POINT('Ctrl Pts',(36.8845452411468,-50.99771444784,40.134683756585));
#168521=CARTESIAN_POINT('Ctrl Pts',(36.8793106050087,-50.9996165178737,
40.1322415082996));
#168522=CARTESIAN_POINT('Ctrl Pts',(36.8609893785252,-51.0062737629917,
40.1236936393009));
#168523=CARTESIAN_POINT('Ctrl Pts',(36.8428672144359,-51.0114266762819,
40.113394140767));
#168524=CARTESIAN_POINT('Ctrl Pts',(36.8253449818068,-51.0150372064713,
40.101665321223));
#168525=CARTESIAN_POINT('Ctrl Pts',(36.8165838654922,-51.0168424715661,
40.095800911451));
#168526=CARTESIAN_POINT('Ctrl Pts',(36.8079727326366,-51.0182621417027,
40.0895791707949));
#168527=CARTESIAN_POINT('Ctrl Pts',(36.7995616970579,-51.0192914676907,
40.0830403822906));
#168528=CARTESIAN_POINT('Ctrl Pts',(36.7953561792686,-51.0198061306846,
40.0797709880385));
#168529=CARTESIAN_POINT('Ctrl Pts',(36.7912006858666,-51.020223207737,40.0764223317514));
#168530=CARTESIAN_POINT('Ctrl Pts',(36.7871014813876,-51.0205421056327,
40.0729994484778));
#168531=CARTESIAN_POINT('Ctrl Pts',(36.7830022769086,-51.0208610035283,
40.0695765652042));
#168532=CARTESIAN_POINT('Ctrl Pts',(36.7789594281949,-51.0210816112667,
40.0660793733488));
#168533=CARTESIAN_POINT('Ctrl Pts',(36.7749790641714,-51.0212035636551,
40.0625130768817));
#168534=CARTESIAN_POINT('Ctrl Pts',(36.7749451200025,-51.0212046036536,
40.0624826638418));
#168535=CARTESIAN_POINT('Ctrl Pts',(36.7749111804867,-51.0212056365644,
40.0624522459912));
#168536=CARTESIAN_POINT('Ctrl Pts',(36.7748772456271,-51.0212066623876,
40.0624218233329));
#168537=CARTESIAN_POINT('Ctrl Pts',(36.7575462174155,-51.0217305652762,
40.0468845275906));
#168538=CARTESIAN_POINT('Ctrl Pts',(36.7413978659072,-51.0205340689292,
40.0302263329253));
#168539=CARTESIAN_POINT('Ctrl Pts',(36.7264984065494,-51.0178063409627,
40.0127515884767));
#168540=CARTESIAN_POINT('Ctrl Pts',(36.7110950573695,-51.0149863630476,
39.9946858597744));
#168541=CARTESIAN_POINT('Ctrl Pts',(36.6970257816922,-51.0105292970939,
39.9757460620525));
#168542=CARTESIAN_POINT('Ctrl Pts',(36.6843954909291,-51.0046027002037,
39.9562444559169));
#168543=CARTESIAN_POINT('Ctrl Pts',(36.6720054548731,-50.9987888396571,
39.9371138113653));
#168544=CARTESIAN_POINT('Ctrl Pts',(36.6609997277928,-50.9915600117749,
39.9174410654397));
#168545=CARTESIAN_POINT('Ctrl Pts',(36.6515157237725,-50.9830457809177,
39.8975196504191));
#168546=CARTESIAN_POINT('Ctrl Pts',(36.645232903603,-50.97740540147,39.8843224113805));
#168547=CARTESIAN_POINT('Ctrl Pts',(36.6396186946846,-50.9712003466848,
39.8710160447147));
#168548=CARTESIAN_POINT('Ctrl Pts',(36.6347241449654,-50.9644637245894,
39.8576902534424));
#168549=CARTESIAN_POINT('',(36.4252947698678,-50.6762142289949,39.2875012672119));
#168550=CARTESIAN_POINT('',(36.6347241449653,-50.9644637245894,39.8576902534424));
#168551=CARTESIAN_POINT('',(31.4795232016789,-53.8880358395971,39.2875012672119));
#168552=CARTESIAN_POINT('Origin',(5.53234440788222E-15,0.,39.2875012672119));
#168553=CARTESIAN_POINT('',(31.6576696180583,-54.1966007261208,39.8576902534424));
#168554=CARTESIAN_POINT('',(31.4795232016789,-53.8880358395971,39.2875012672119));
#168555=CARTESIAN_POINT('',(31.4902932482907,-54.5122556166612,40.1599502534424));
#168556=CARTESIAN_POINT('Ctrl Pts',(31.6576696180583,-54.1966007261208,
39.8576902534424));
#168557=CARTESIAN_POINT('Ctrl Pts',(31.6638224711874,-54.2072580443422,
39.8773836120376));
#168558=CARTESIAN_POINT('Ctrl Pts',(31.6682661704393,-54.2188555266763,
39.8969946442155));
#168559=CARTESIAN_POINT('Ctrl Pts',(31.6709833936515,-54.231205042323,39.9162525288275));
#168560=CARTESIAN_POINT('Ctrl Pts',(31.67375521647,-54.2438027078788,39.9358973794106));
#168561=CARTESIAN_POINT('Ctrl Pts',(31.6747309854167,-54.2571837147331,
39.9551762199791));
#168562=CARTESIAN_POINT('Ctrl Pts',(31.6738510973601,-54.2711824151086,
39.9738152034302));
#168563=CARTESIAN_POINT('Ctrl Pts',(31.673005392157,-54.2846372786644,39.9917300792704));
#168564=CARTESIAN_POINT('Ctrl Pts',(31.6704454915893,-54.2986636530715,
40.0090551158181));
#168565=CARTESIAN_POINT('Ctrl Pts',(31.6660771734232,-54.3131329740911,
40.0255394551594));
#168566=CARTESIAN_POINT('Ctrl Pts',(31.6627215829929,-54.3242478043989,
40.0382021526188));
#168567=CARTESIAN_POINT('Ctrl Pts',(31.6582981215823,-54.3356244578591,
40.0503687782141));
#168568=CARTESIAN_POINT('Ctrl Pts',(31.6527458376967,-54.3472079546994,
40.0619155352442));
#168569=CARTESIAN_POINT('Ctrl Pts',(31.6527312861508,-54.3472383129789,
40.0619457972351));
#168570=CARTESIAN_POINT('Ctrl Pts',(31.6527167260613,-54.3472686729569,
40.0619760547305));
#168571=CARTESIAN_POINT('Ctrl Pts',(31.6527021574293,-54.3472990346305,
40.0620063077269));
#168572=CARTESIAN_POINT('Ctrl Pts',(31.6511401038187,-54.3505544234701,
40.06525004417));
#168573=CARTESIAN_POINT('Ctrl Pts',(31.6494796970076,-54.3538274103384,
40.0684393223556));
#168574=CARTESIAN_POINT('Ctrl Pts',(31.6477231007679,-54.3571135597833,
40.0715697951759));
#168575=CARTESIAN_POINT('Ctrl Pts',(31.6379480420923,-54.3754002342707,
40.0889901646433));
#168576=CARTESIAN_POINT('Ctrl Pts',(31.6251987170214,-54.3940968201805,
40.1045963098266));
#168577=CARTESIAN_POINT('Ctrl Pts',(31.6099016141331,-54.4124255228592,
40.1176634650754));
#168578=CARTESIAN_POINT('Ctrl Pts',(31.6030360625191,-54.4206516984414,
40.123528185308));
#168579=CARTESIAN_POINT('Ctrl Pts',(31.5956573884055,-54.4288041214182,
40.1288820140928));
#168580=CARTESIAN_POINT('Ctrl Pts',(31.5878037911381,-54.4368146919236,
40.1336621774101));
#168581=CARTESIAN_POINT('Ctrl Pts',(31.5843907239925,-54.4402959775153,
40.1357395717319));
#168582=CARTESIAN_POINT('Ctrl Pts',(31.58088799234,-54.4437502703989,40.1377083672883));
#168583=CARTESIAN_POINT('Ctrl Pts',(31.5772987574368,-54.4471718528272,
40.1395632548791));
#168584=CARTESIAN_POINT('Ctrl Pts',(31.5647364352753,-54.4591473913263,
40.1460553614469));
#168585=CARTESIAN_POINT('Ctrl Pts',(31.5511144466741,-54.4707222239581,
40.151152097463));
#168586=CARTESIAN_POINT('Ctrl Pts',(31.5365683393825,-54.4816512176785,
40.1546258197409));
#168587=CARTESIAN_POINT('Ctrl Pts',(31.5292952857367,-54.4871157145387,
40.1563626808798));
#168588=CARTESIAN_POINT('Ctrl Pts',(31.5217912027244,-54.4924187521963,
40.1576937882008));
#168589=CARTESIAN_POINT('Ctrl Pts',(31.5140730377804,-54.4975296958773,
40.1585906813668));
#168590=CARTESIAN_POINT('Ctrl Pts',(31.5102139553083,-54.5000851677177,
40.1590391279498));
#168591=CARTESIAN_POINT('Ctrl Pts',(31.5063013524149,-54.5025926161708,
40.1593790209175));
#168592=CARTESIAN_POINT('Ctrl Pts',(31.5023373478779,-54.5050482124961,
40.1596068022931));
#168593=CARTESIAN_POINT('Ctrl Pts',(31.4983733433408,-54.5075038088215,
40.1598345836687));
#168594=CARTESIAN_POINT('Ctrl Pts',(31.4943579363066,-54.5099075515417,
40.1599502506865));
#168595=CARTESIAN_POINT('Ctrl Pts',(31.4902932482907,-54.5122556166611,
40.1599502534424));
#168596=CARTESIAN_POINT('',(31.4638515574739,-54.527521733972,40.1599502534424));
#168597=CARTESIAN_POINT('Origin',(5.57749365020894E-15,5.82947588787858E-15,
40.1599502534424));
#168598=CARTESIAN_POINT('',(31.1067982185534,-54.5146464769138,39.8576902534424));
#168599=CARTESIAN_POINT('Ctrl Pts',(31.4638515574739,-54.527521733972,40.1599502534424));
#168600=CARTESIAN_POINT('Ctrl Pts',(31.4605414731919,-54.5294317356858,
40.1599502447858));
#168601=CARTESIAN_POINT('Ctrl Pts',(31.457216601512,-54.5312951627228,40.1598744685927));
#168602=CARTESIAN_POINT('Ctrl Pts',(31.4538791743432,-54.533112022376,40.1597246934279));
#168603=CARTESIAN_POINT('Ctrl Pts',(31.434592962471,-54.5436112298318,40.1588591777434));
#168604=CARTESIAN_POINT('Ctrl Pts',(31.4148859438252,-54.5525583311782,
40.1555254706017));
#168605=CARTESIAN_POINT('Ctrl Pts',(31.3951944477259,-54.5599504658514,
40.1500631826373));
#168606=CARTESIAN_POINT('Ctrl Pts',(31.3872524143686,-54.5629318838127,
40.1478601162475));
#168607=CARTESIAN_POINT('Ctrl Pts',(31.3793127123318,-54.5656607810288,
40.1453112228303));
#168608=CARTESIAN_POINT('Ctrl Pts',(31.3714030065917,-54.5681385507008,
40.1424401896328));
#168609=CARTESIAN_POINT('Ctrl Pts',(31.3684848053917,-54.5690526972782,
40.1413809526905));
#168610=CARTESIAN_POINT('Ctrl Pts',(31.3655707565305,-54.569932546879,40.1402777640511));
#168611=CARTESIAN_POINT('Ctrl Pts',(31.3626622846451,-54.5707781137755,
40.1391317641987));
#168612=CARTESIAN_POINT('Ctrl Pts',(31.3572088998598,-54.5723635517063,
40.1369830144753));
#168613=CARTESIAN_POINT('Ctrl Pts',(31.3517751216268,-54.5738284644992,
40.1346837565849));
#168614=CARTESIAN_POINT('Ctrl Pts',(31.3463703409154,-54.5751729463229,
40.1322415082996));
#168615=CARTESIAN_POINT('Ctrl Pts',(31.3274536084258,-54.579878632706,40.1236936393008));
#168616=CARTESIAN_POINT('Ctrl Pts',(31.30889209334,-54.5831090358348,40.113394140767));
#168617=CARTESIAN_POINT('Ctrl Pts',(31.2910884461624,-54.5848682151123,
40.101665321223));
#168618=CARTESIAN_POINT('Ctrl Pts',(31.2821866225735,-54.5857478047511,
40.095800911451));
#168619=CARTESIAN_POINT('Ctrl Pts',(31.273474266467,-54.5862595893019,40.0895791707949));
#168620=CARTESIAN_POINT('Ctrl Pts',(31.2650017135576,-54.5864040839108,
40.0830403822906));
#168621=CARTESIAN_POINT('Ctrl Pts',(31.2607654371028,-54.5864763312152,
40.0797709880385));
#168622=CARTESIAN_POINT('Ctrl Pts',(31.2565891115051,-54.5864567561364,
40.0764223317514));
#168623=CARTESIAN_POINT('Ctrl Pts',(31.2524790289902,-54.5863454235313,
40.0729994484778));
#168624=CARTESIAN_POINT('Ctrl Pts',(31.2483689464753,-54.5862340909261,
40.0695765652042));
#168625=CARTESIAN_POINT('Ctrl Pts',(31.244325185122,-54.5860308973889,40.0660793733488));
#168626=CARTESIAN_POINT('Ctrl Pts',(31.2403538784534,-54.5857361203748,
40.0625130768817));
#168627=CARTESIAN_POINT('Ctrl Pts',(31.2403200115247,-54.5857336065442,
40.0624826638418));
#168628=CARTESIAN_POINT('Ctrl Pts',(31.2402861499645,-54.5857310861512,
40.0624522459912));
#168629=CARTESIAN_POINT('Ctrl Pts',(31.240252293776,-54.5857285591961,40.0624218233329));
#168630=CARTESIAN_POINT('Ctrl Pts',(31.2229614439864,-54.584438006344,40.0468845275906));
#168631=CARTESIAN_POINT('Ctrl Pts',(31.2070266227617,-54.5815601021618,
40.0302263329253));
#168632=CARTESIAN_POINT('Ctrl Pts',(31.1924939094138,-54.5772898993843,
40.0127515884768));
#168633=CARTESIAN_POINT('Ctrl Pts',(31.1774697093504,-54.5728752811845,
39.9946858597746));
#168634=CARTESIAN_POINT('Ctrl Pts',(31.1639433968922,-54.5669719917386,
39.9757460620528));
#168635=CARTESIAN_POINT('Ctrl Pts',(31.1520017942489,-54.5597576364823,
39.9562444559174));
#168636=CARTESIAN_POINT('Ctrl Pts',(31.1402873460154,-54.5526805134434,
39.9371138113662));
#168637=CARTESIAN_POINT('Ctrl Pts',(31.1300975277295,-54.544340874098,39.9174410654408));
#168638=CARTESIAN_POINT('Ctrl Pts',(31.1215554575431,-54.5348819367227,
39.8975196504205));
#168639=CARTESIAN_POINT('Ctrl Pts',(31.1158966355154,-54.5286157223262,
39.8843224113815));
#168640=CARTESIAN_POINT('Ctrl Pts',(31.1109617866619,-54.5218578148494,
39.8710160447152));
#168641=CARTESIAN_POINT('Ctrl Pts',(31.1067982185534,-54.5146464769138,
39.8576902534424));
#168642=CARTESIAN_POINT('',(30.9286463962977,-54.2060847114742,39.2875012672119));
#168643=CARTESIAN_POINT('',(31.1067982185534,-54.5146464769138,39.8576902534424));
#168644=CARTESIAN_POINT('',(25.6742415049979,-56.8833377255395,39.2875012672119));
#168645=CARTESIAN_POINT('Origin',(5.53234440788222E-15,0.,39.2875012672119));
#168646=CARTESIAN_POINT('',(25.8191582032619,-57.2088336324699,39.8576902534424));
#168647=CARTESIAN_POINT('',(25.6742415049979,-56.8833377255395,39.2875012672119));
#168648=CARTESIAN_POINT('',(25.6197038181297,-57.5052637377732,40.1599502534424));
#168649=CARTESIAN_POINT('Ctrl Pts',(25.8191582032619,-57.2088336324699,
39.8576902534424));
#168650=CARTESIAN_POINT('Ctrl Pts',(25.8241633573212,-57.2200757170683,
39.8773836120359));
#168651=CARTESIAN_POINT('Ctrl Pts',(25.8273704465175,-57.2320741602337,
39.8969946442123));
#168652=CARTESIAN_POINT('Ctrl Pts',(25.8287819086041,-57.2446400511071,
39.9162525288227));
#168653=CARTESIAN_POINT('Ctrl Pts',(25.8302217324661,-57.2574584397114,
39.9358973794043));
#168654=CARTESIAN_POINT('Ctrl Pts',(25.8297934599654,-57.2708681396374,
39.9551762199714));
#168655=CARTESIAN_POINT('Ctrl Pts',(25.8274551293905,-57.2846981803199,
39.9738152034211));
#168656=CARTESIAN_POINT('Ctrl Pts',(25.8252076408387,-57.297990936459,39.9917300792603));
#168657=CARTESIAN_POINT('Ctrl Pts',(25.8211956083131,-57.3116728904459,
40.0090551158071));
#168658=CARTESIAN_POINT('Ctrl Pts',(25.8153387643616,-57.325606333425,40.0255394551476));
#168659=CARTESIAN_POINT('Ctrl Pts',(25.8108397400745,-57.3363095208216,
40.0382021526112));
#168660=CARTESIAN_POINT('Ctrl Pts',(25.8052513267436,-57.3471614741636,
40.0503687782105));
#168661=CARTESIAN_POINT('Ctrl Pts',(25.798518653724,-57.3581011436975,40.0619155352442));
#168662=CARTESIAN_POINT('Ctrl Pts',(25.7985010085887,-57.3581298146203,
40.0619457972351));
#168663=CARTESIAN_POINT('Ctrl Pts',(25.798483354779,-57.3581584863394,40.0619760547305));
#168664=CARTESIAN_POINT('Ctrl Pts',(25.7984656922965,-57.3581871588519,
40.0620063077269));
#168665=CARTESIAN_POINT('Ctrl Pts',(25.7965719149862,-57.3612614352674,
40.06525004417));
#168666=CARTESIAN_POINT('Ctrl Pts',(25.7945784837697,-57.3643429325988,
40.0684393223556));
#168667=CARTESIAN_POINT('Ctrl Pts',(25.7924880141965,-57.3674274658676,
40.0715697951759));
#168668=CARTESIAN_POINT('Ctrl Pts',(25.7808550263334,-57.384592192176,40.0889901646422));
#168669=CARTESIAN_POINT('Ctrl Pts',(25.7662212180069,-57.4018536888734,
40.1045963098245));
#168670=CARTESIAN_POINT('Ctrl Pts',(25.7490920431255,-57.4184830023427,
40.1176634650729));
#168671=CARTESIAN_POINT('Ctrl Pts',(25.7414042322284,-57.4259464685158,
40.1235281853064));
#168672=CARTESIAN_POINT('Ctrl Pts',(25.7332138190169,-57.4332829502016,
40.1288820140921));
#168673=CARTESIAN_POINT('Ctrl Pts',(25.724565911951,-57.4404287135112,40.1336621774101));
#168674=CARTESIAN_POINT('Ctrl Pts',(25.7208076485112,-57.4435341655924,
40.1357395717319));
#168675=CARTESIAN_POINT('Ctrl Pts',(25.7169630332624,-57.4466034003412,
40.1377083672884));
#168676=CARTESIAN_POINT('Ctrl Pts',(25.7130358078103,-57.4496310617743,
40.1395632548792));
#168677=CARTESIAN_POINT('Ctrl Pts',(25.699290518728,-57.4602278767899,40.146055361447));
#168678=CARTESIAN_POINT('Ctrl Pts',(25.6845332533381,-57.4703154157423,
40.1511520974629));
#168679=CARTESIAN_POINT('Ctrl Pts',(25.6689244402255,-57.4796640570498,
40.1546258197408));
#168680=CARTESIAN_POINT('Ctrl Pts',(25.6611200336693,-57.4843383777036,
40.1563626808798));
#168681=CARTESIAN_POINT('Ctrl Pts',(25.6531027404319,-57.4888279745006,
40.1576937882008));
#168682=CARTESIAN_POINT('Ctrl Pts',(25.6448926173141,-57.4931041519764,
40.1585906813668));
#168683=CARTESIAN_POINT('Ctrl Pts',(25.6407875557553,-57.4952422407143,
40.1590391279498));
#168684=CARTESIAN_POINT('Ctrl Pts',(25.6366342867764,-57.4973269747345,
40.1593790209175));
#168685=CARTESIAN_POINT('Ctrl Pts',(25.6324353177606,-57.4993547677436,
40.1596068022931));
#168686=CARTESIAN_POINT('Ctrl Pts',(25.6282363487449,-57.5013825607528,
40.1598345836687));
#168687=CARTESIAN_POINT('Ctrl Pts',(25.6239916789979,-57.5033534111922,
40.1599502506864));
#168688=CARTESIAN_POINT('Ctrl Pts',(25.6197038181297,-57.5052637377733,
40.1599502534424));
#168689=CARTESIAN_POINT('',(25.5918112338793,-57.5176823163889,40.1599502534424));
#168690=CARTESIAN_POINT('Origin',(5.59198795571863E-15,5.83686110540852E-15,
40.1599502534424));
#168691=CARTESIAN_POINT('',(25.2380597013429,-57.4675553545141,39.8576902534424));
#168692=CARTESIAN_POINT('Ctrl Pts',(25.5918112338793,-57.5176823163889,
40.1599502534424));
#168693=CARTESIAN_POINT('Ctrl Pts',(25.5883196330413,-57.5192358568901,
40.1599502447858));
#168694=CARTESIAN_POINT('Ctrl Pts',(25.5848181941918,-57.5207415321516,
40.1598744685927));
#168695=CARTESIAN_POINT('Ctrl Pts',(25.5813091362507,-57.5221995827243,
40.1597246934279));
#168696=CARTESIAN_POINT('Ctrl Pts',(25.5610311102425,-57.5306253163346,
40.1588591777434));
#168697=CARTESIAN_POINT('Ctrl Pts',(25.5404968219507,-57.5374634601495,
40.1555254706012));
#168698=CARTESIAN_POINT('Ctrl Pts',(25.5201405094481,-57.5427567781089,
40.1500631826359));
#168699=CARTESIAN_POINT('Ctrl Pts',(25.5119303403444,-57.5448916950081,
40.1478601162464));
#168700=CARTESIAN_POINT('Ctrl Pts',(25.5037488853954,-57.5467757181865,
40.1453112228297));
#168701=CARTESIAN_POINT('Ctrl Pts',(25.4956235123965,-57.5484131249908,
40.1424401896328));
#168702=CARTESIAN_POINT('Ctrl Pts',(25.492625743071,-57.5490172286906,40.1413809526905));
#168703=CARTESIAN_POINT('Ctrl Pts',(25.4896356883477,-57.5495876573339,
40.1402777640511));
#168704=CARTESIAN_POINT('Ctrl Pts',(25.4866547635673,-57.5501245740298,
40.1391317641987));
#168705=CARTESIAN_POINT('Ctrl Pts',(25.481065529604,-57.5511312928345,40.1369830144753));
#168706=CARTESIAN_POINT('Ctrl Pts',(25.4755083930936,-57.5520201961934,
40.1346837565849));
#168707=CARTESIAN_POINT('Ctrl Pts',(25.4699926837176,-57.552792359383,40.1322415082996));
#168708=CARTESIAN_POINT('Ctrl Pts',(25.4506877009016,-57.5554949305466,
40.1236936393008));
#168709=CARTESIAN_POINT('Ctrl Pts',(25.4318901986628,-57.5567674305411,
40.113394140767));
#168710=CARTESIAN_POINT('Ctrl Pts',(25.4140001974206,-57.5566559849705,
40.101665321223));
#168711=CARTESIAN_POINT('Ctrl Pts',(25.4050551967996,-57.5566002621852,
40.095800911451));
#168712=CARTESIAN_POINT('Ctrl Pts',(25.3963370718388,-57.5561985539314,
40.0895791707949));
#168713=CARTESIAN_POINT('Ctrl Pts',(25.3878958286612,-57.5554566340481,
40.0830403822906));
#168714=CARTESIAN_POINT('Ctrl Pts',(25.3836752070724,-57.5550856741065,
40.0797709880385));
#168715=CARTESIAN_POINT('Ctrl Pts',(25.3795238059763,-57.5546296613652,
40.0764223317514));
#168716=CARTESIAN_POINT('Ctrl Pts',(25.3754478763495,-57.5540893180425,
40.0729994484778));
#168717=CARTESIAN_POINT('Ctrl Pts',(25.3713719467228,-57.5535489747198,
40.0695765652042));
#168718=CARTESIAN_POINT('Ctrl Pts',(25.3673715770255,-57.552924206138,40.0660793733488));
#168719=CARTESIAN_POINT('Ctrl Pts',(25.3634528381786,-57.55221592936,40.0625130768817));
#168720=CARTESIAN_POINT('Ctrl Pts',(25.3634194195433,-57.5522098892424,
40.0624826638418));
#168721=CARTESIAN_POINT('Ctrl Pts',(25.3633860069332,-57.5522038431595,
40.0624522459912));
#168722=CARTESIAN_POINT('Ctrl Pts',(25.3633526003511,-57.552197791112,40.0624218233329));
#168723=CARTESIAN_POINT('Ctrl Pts',(25.3462913711534,-57.5491069220866,
40.0468845275917));
#168724=CARTESIAN_POINT('Ctrl Pts',(25.3307446654493,-57.54457914099,40.0302263329276));
#168725=CARTESIAN_POINT('Ctrl Pts',(25.3167379215606,-57.5388132486373,
40.0127515884805));
#168726=CARTESIAN_POINT('Ctrl Pts',(25.3022574788943,-57.532852357634,39.9946858597797));
#168727=CARTESIAN_POINT('Ctrl Pts',(25.2894223267656,-57.5255675223713,
39.9757460620594));
#168728=CARTESIAN_POINT('Ctrl Pts',(25.2783002469397,-57.5171444507355,
39.9562444559255));
#168729=CARTESIAN_POINT('Ctrl Pts',(25.2673897324753,-57.5088816036461,
39.9371138113757));
#168730=CARTESIAN_POINT('Ctrl Pts',(25.2581274647651,-57.4995225236723,
39.9174410654518));
#168731=CARTESIAN_POINT('Ctrl Pts',(25.2506209171206,-57.4892225138769,
39.8975196504329));
#168732=CARTESIAN_POINT('Ctrl Pts',(25.2456480924715,-57.4823991184863,
39.8843224113898));
#168733=CARTESIAN_POINT('Ctrl Pts',(25.2414466709183,-57.4751623993644,
39.8710160447193));
#168734=CARTESIAN_POINT('Ctrl Pts',(25.2380597013429,-57.4675553545141,
39.8576902534424));
#168735=CARTESIAN_POINT('',(25.0931373005745,-57.1420619865022,39.2875012672119));
#168736=CARTESIAN_POINT('',(25.2380597013429,-57.4675553545141,39.8576902534424));
#168737=CARTESIAN_POINT('',(19.5876674457077,-59.2554138597572,39.2875012672119));
#168738=CARTESIAN_POINT('Origin',(5.53234440788222E-15,0.,39.2875012672119));
#168739=CARTESIAN_POINT('',(19.6977666881844,-59.5942745858236,39.8576902534424));
#168740=CARTESIAN_POINT('',(19.5876674457077,-59.2554138597572,39.2875012672119));
#168741=CARTESIAN_POINT('',(19.4684195516695,-59.8682321556242,40.1599502534424));
#168742=CARTESIAN_POINT('Ctrl Pts',(19.6977666881844,-59.5942745858236,
39.8576902534424));
#168743=CARTESIAN_POINT('Ctrl Pts',(19.7015693056589,-59.6059782661672,
39.8773836120338));
#168744=CARTESIAN_POINT('Ctrl Pts',(19.7035046472594,-59.6182462127093,
39.8969946442081));
#168745=CARTESIAN_POINT('Ctrl Pts',(19.7035948839469,-59.6308908042792,
39.9162525288166));
#168746=CARTESIAN_POINT('Ctrl Pts',(19.7036869338411,-59.6437894749839,
39.9358973793963));
#168747=CARTESIAN_POINT('Ctrl Pts',(19.7018593121365,-59.6570809485028,
39.9551762199616));
#168748=CARTESIAN_POINT('Ctrl Pts',(19.6980881582828,-59.6705908046724,
39.9738152034098));
#168749=CARTESIAN_POINT('Ctrl Pts',(19.6944635103376,-59.683575815177,39.9917300792478));
#168750=CARTESIAN_POINT('Ctrl Pts',(19.6890433025225,-59.6967634463928,
40.0090551157937));
#168751=CARTESIAN_POINT('Ctrl Pts',(19.6817621015939,-59.7100083536145,
40.0255394551334));
#168752=CARTESIAN_POINT('Ctrl Pts',(19.6761689357006,-59.7201826317395,
40.0382021526021));
#168753=CARTESIAN_POINT('Ctrl Pts',(19.6694767982743,-59.7303909886918,
40.0503687782062));
#168754=CARTESIAN_POINT('Ctrl Pts',(19.661637500694,-59.7405669736108,40.0619155352442));
#168755=CARTESIAN_POINT('Ctrl Pts',(19.6616169552931,-59.7405936430524,
40.0619457972351));
#168756=CARTESIAN_POINT('Ctrl Pts',(19.6615964011821,-59.7406203123793,
40.0619760547305));
#168757=CARTESIAN_POINT('Ctrl Pts',(19.6615758383628,-59.7406469815886,
40.0620063077269));
#168758=CARTESIAN_POINT('Ctrl Pts',(19.6593710859735,-59.7435064631642,
40.06525004417));
#168759=CARTESIAN_POINT('Ctrl Pts',(19.6570664708011,-59.7463627094291,
40.0684393223557));
#168760=CARTESIAN_POINT('Ctrl Pts',(19.6546650315164,-59.74921183173,40.0715697951759));
#168761=CARTESIAN_POINT('Ctrl Pts',(19.6413015679154,-59.7650665495262,
40.0889901646412));
#168762=CARTESIAN_POINT('Ctrl Pts',(19.6249436073997,-59.7807038364415,
40.1045963098227));
#168763=CARTESIAN_POINT('Ctrl Pts',(19.6061700313499,-59.7954515664635,
40.1176634650705));
#168764=CARTESIAN_POINT('Ctrl Pts',(19.5977441904346,-59.80207055193,40.123528185305));
#168765=CARTESIAN_POINT('Ctrl Pts',(19.5888317740061,-59.8085107122958,
40.1288820140915));
#168766=CARTESIAN_POINT('Ctrl Pts',(19.5794843054211,-59.814713377931,40.1336621774101));
#168767=CARTESIAN_POINT('Ctrl Pts',(19.5754220220079,-59.8174089725188,
40.1357395717319));
#168768=CARTESIAN_POINT('Ctrl Pts',(19.571277645572,-59.8200595219548,40.1377083672883));
#168769=CARTESIAN_POINT('Ctrl Pts',(19.5670554570749,-59.8226600907003,
40.1395632548791));
#168770=CARTESIAN_POINT('Ctrl Pts',(19.5522777973353,-59.8317620813095,
40.1460553614469));
#168771=CARTESIAN_POINT('Ctrl Pts',(19.5365469388443,-59.8402518053948,
40.1511520974629));
#168772=CARTESIAN_POINT('Ctrl Pts',(19.5200464333337,-59.847917668619,40.1546258197408));
#168773=CARTESIAN_POINT('Ctrl Pts',(19.5117961805784,-59.8517506002311,
40.1563626808798));
#168774=CARTESIAN_POINT('Ctrl Pts',(19.5033535162583,-59.8553775672055,
40.1576937882008));
#168775=CARTESIAN_POINT('Ctrl Pts',(19.4947413867939,-59.858772127781,40.1585906813668));
#168776=CARTESIAN_POINT('Ctrl Pts',(19.4904353220616,-59.8604694080687,
40.1590391279498));
#168777=CARTESIAN_POINT('Ctrl Pts',(19.4860868910813,-59.8621085868739,
40.1593790209175));
#168778=CARTESIAN_POINT('Ctrl Pts',(19.4816989623701,-59.8636863596422,
40.1596068022931));
#168779=CARTESIAN_POINT('Ctrl Pts',(19.4773110336589,-59.8652641324105,
40.1598345836687));
#168780=CARTESIAN_POINT('Ctrl Pts',(19.4728836066891,-59.8667804975193,
40.1599502506865));
#168781=CARTESIAN_POINT('Ctrl Pts',(19.4684195516695,-59.8682321556242,
40.1599502534424));
#168782=CARTESIAN_POINT('',(19.4393816709755,-59.8776671349986,40.1599502534424));
#168783=CARTESIAN_POINT('Origin',(5.60717482534548E-15,5.84269079846304E-15,
40.1599502534424));
#168784=CARTESIAN_POINT('',(19.092807720641,-59.7908376697912,39.8576902534424));
#168785=CARTESIAN_POINT('Ctrl Pts',(19.4393816709755,-59.8776671349986,
40.1599502534424));
#168786=CARTESIAN_POINT('Ctrl Pts',(19.435746808291,-59.8788471933725,40.1599502447858));
#168787=CARTESIAN_POINT('Ctrl Pts',(19.4321071647686,-59.8799786203651,
40.1598744685927));
#168788=CARTESIAN_POINT('Ctrl Pts',(19.4284649220283,-59.8810618871501,
40.1597246934279));
#168789=CARTESIAN_POINT('Ctrl Pts',(19.4074172521856,-59.8873218328123,
40.1588591777435));
#168790=CARTESIAN_POINT('Ctrl Pts',(19.3862806722126,-59.89197609896,40.1555254706023));
#168791=CARTESIAN_POINT('Ctrl Pts',(19.3654825713311,-59.8951126055061,
40.1500631826386));
#168792=CARTESIAN_POINT('Ctrl Pts',(19.3570942188067,-59.8963776307482,
40.1478601162485));
#168793=CARTESIAN_POINT('Ctrl Pts',(19.3487606486729,-59.897396138138,40.1453112228309));
#168794=CARTESIAN_POINT('Ctrl Pts',(19.3405086316971,-59.8981752423037,
40.1424401896328));
#168795=CARTESIAN_POINT('Ctrl Pts',(19.3374641384343,-59.8984626844394,
40.1413809526906));
#168796=CARTESIAN_POINT('Ctrl Pts',(19.3344308375141,-59.8987174423897,
40.1402777640511));
#168797=CARTESIAN_POINT('Ctrl Pts',(19.3314101194744,-59.8989398263133,
40.1391317641987));
#168798=CARTESIAN_POINT('Ctrl Pts',(19.3257462731499,-59.89935679617,40.1369830144753));
#168799=CARTESIAN_POINT('Ctrl Pts',(19.3201266635127,-59.8996599510837,
40.1346837565849));
#168800=CARTESIAN_POINT('Ctrl Pts',(19.3145604567382,-59.8998513356576,
40.1322415082996));
#168801=CARTESIAN_POINT('Ctrl Pts',(19.2950787330274,-59.9005211816664,
40.1236936393008));
#168802=CARTESIAN_POINT('Ctrl Pts',(19.2762511930037,-59.8998218367506,
40.113394140767));
#168803=CARTESIAN_POINT('Ctrl Pts',(19.2584708442944,-59.8978409873527,
40.101665321223));
#168804=CARTESIAN_POINT('Ctrl Pts',(19.2495806699398,-59.8968505626538,
40.095800911451));
#168805=CARTESIAN_POINT('Ctrl Pts',(19.2409522937263,-59.8955397627951,
40.0895791707949));
#168806=CARTESIAN_POINT('Ctrl Pts',(19.2326348443073,-59.8939195570492,
40.0830403822906));
#168807=CARTESIAN_POINT('Ctrl Pts',(19.2284761195978,-59.8931094541763,
40.0797709880385));
#168808=CARTESIAN_POINT('Ctrl Pts',(19.2243951266223,-59.8922219999435,
40.0764223317514));
#168809=CARTESIAN_POINT('Ctrl Pts',(19.2203980066217,-59.8912585660178,
40.0729994484778));
#168810=CARTESIAN_POINT('Ctrl Pts',(19.2164008866211,-59.8902951320921,
40.0695765652042));
#168811=CARTESIAN_POINT('Ctrl Pts',(19.2124877374673,-59.889255633561,40.0660793733488));
#168812=CARTESIAN_POINT('Ctrl Pts',(19.208664500965,-59.8881416170476,40.0625130768817));
#168813=CARTESIAN_POINT('Ctrl Pts',(19.2086318967648,-59.8881321168199,
40.0624826638418));
#168814=CARTESIAN_POINT('Ctrl Pts',(19.2085992991801,-59.8881226112892,
40.0624522459912));
#168815=CARTESIAN_POINT('Ctrl Pts',(19.208566708214,-59.8881131004568,40.0624218233329));
#168816=CARTESIAN_POINT('Ctrl Pts',(19.1919220260051,-59.883255779466,40.0468845275922));
#168817=CARTESIAN_POINT('Ctrl Pts',(19.176933768782,-59.8771277287721,40.0302263329289));
#168818=CARTESIAN_POINT('Ctrl Pts',(19.1636064551692,-59.8699293191674,
40.0127515884825));
#168819=CARTESIAN_POINT('Ctrl Pts',(19.1498284206597,-59.8624874641298,
39.9946858597826));
#168820=CARTESIAN_POINT('Ctrl Pts',(19.1378250534729,-59.8539008972296,
39.9757460620633));
#168821=CARTESIAN_POINT('Ctrl Pts',(19.1276443522982,-59.8443613941496,
39.9562444559305));
#168822=CARTESIAN_POINT('Ctrl Pts',(19.1176573094822,-59.8350033524913,
39.9371138113817));
#168823=CARTESIAN_POINT('Ctrl Pts',(19.109424071691,-59.8247273719274,39.9174410654588));
#168824=CARTESIAN_POINT('Ctrl Pts',(19.1030352898953,-59.8136991387744,
39.8975196504409));
#168825=CARTESIAN_POINT('Ctrl Pts',(19.0988029459332,-59.8063933209376,
39.8843224113952));
#168826=CARTESIAN_POINT('Ctrl Pts',(19.0953809833349,-59.7987570771804,
39.871016044722));
#168827=CARTESIAN_POINT('Ctrl Pts',(19.092807720641,-59.7908376697912,39.8576902534424));
#168828=CARTESIAN_POINT('',(18.9827025415095,-59.4519788726608,39.2875012672119));
#168829=CARTESIAN_POINT('',(19.092807720641,-59.7908376697912,39.8576902534424));
#168830=CARTESIAN_POINT('',(13.2864868028994,-60.9782752797348,39.2875012672119));
#168831=CARTESIAN_POINT('Origin',(5.53234440788222E-15,0.,39.2875012672119));
#168832=CARTESIAN_POINT('',(13.3605623192485,-61.3267881959113,39.8576902534424));
#168833=CARTESIAN_POINT('',(13.2864868028994,-60.9782752797348,39.2875012672119));
#168834=CARTESIAN_POINT('',(13.1038352065726,-61.5752716937452,40.1599502534424));
#168835=CARTESIAN_POINT('Ctrl Pts',(13.3605623192485,-61.3267881959113,
39.8576902534424));
#168836=CARTESIAN_POINT('Ctrl Pts',(13.3631207378657,-61.338825244031,39.8773836120348));
#168837=CARTESIAN_POINT('Ctrl Pts',(13.3637631278628,-61.3512282837623,
39.8969946442099));
#168838=CARTESIAN_POINT('Ctrl Pts',(13.3625311504986,-61.3638130392394,
39.9162525288192));
#168839=CARTESIAN_POINT('Ctrl Pts',(13.3612744179067,-61.3766506715109,
39.9358973793998));
#168840=CARTESIAN_POINT('Ctrl Pts',(13.3580674708032,-61.3896782944596,
39.9551762199659));
#168841=CARTESIAN_POINT('Ctrl Pts',(13.3529048112199,-61.402719949307,39.9738152034148));
#168842=CARTESIAN_POINT('Ctrl Pts',(13.3479427162813,-61.4152549476863,
39.9917300792534));
#168843=CARTESIAN_POINT('Ctrl Pts',(13.341173718106,-61.4278037696855,40.0090551157998));
#168844=CARTESIAN_POINT('Ctrl Pts',(13.3325479345591,-61.4402150271762,
40.0255394551399));
#168845=CARTESIAN_POINT('Ctrl Pts',(13.3259219069573,-61.4497489245038,
40.0382021526063));
#168846=CARTESIAN_POINT('Ctrl Pts',(13.3181993658965,-61.4592018401658,
40.0503687782082));
#168847=CARTESIAN_POINT('Ctrl Pts',(13.3093393327442,-61.4685026502439,
40.0619155352442));
#168848=CARTESIAN_POINT('Ctrl Pts',(13.3093161121774,-61.4685270260084,
40.0619457972351));
#168849=CARTESIAN_POINT('Ctrl Pts',(13.3092928829602,-61.4685514007482,
40.0619760547305));
#168850=CARTESIAN_POINT('Ctrl Pts',(13.3092696450948,-61.4685757744609,
40.0620063077269));
#168851=CARTESIAN_POINT('Ctrl Pts',(13.3067780733549,-61.4711891321181,
40.06525004417));
#168852=CARTESIAN_POINT('Ctrl Pts',(13.3041875240728,-61.4737888336847,
40.0684393223557));
#168853=CARTESIAN_POINT('Ctrl Pts',(13.301501425748,-61.4763713294375,40.0715697951759));
#168854=CARTESIAN_POINT('Ctrl Pts',(13.2865538993123,-61.4907423311162,
40.0889901646409));
#168855=CARTESIAN_POINT('Ctrl Pts',(13.2686510078454,-61.5045840828626,
40.1045963098221));
#168856=CARTESIAN_POINT('Ctrl Pts',(13.248438717854,-61.5172886502217,40.1176634650698));
#168857=CARTESIAN_POINT('Ctrl Pts',(13.2393671621973,-61.5229906359909,
40.1235281853046));
#168858=CARTESIAN_POINT('Ctrl Pts',(13.2298303888519,-61.5284639152914,
40.1288820140913));
#168859=CARTESIAN_POINT('Ctrl Pts',(13.2198857715704,-61.5336555255488,
40.1336621774101));
#168860=CARTESIAN_POINT('Ctrl Pts',(13.2155639754109,-61.5359117291449,
40.1357395717319));
#168861=CARTESIAN_POINT('Ctrl Pts',(13.2111652444434,-61.5381145532937,
40.1377083672884));
#168862=CARTESIAN_POINT('Ctrl Pts',(13.2066943520821,-61.5402595369763,
40.1395632548792));
#168863=CARTESIAN_POINT('Ctrl Pts',(13.1910462288177,-61.5477669798653,
40.146055361447));
#168864=CARTESIAN_POINT('Ctrl Pts',(13.1745141278033,-61.5545658738898,
40.1511520974629));
#168865=CARTESIAN_POINT('Ctrl Pts',(13.1573027128859,-61.560464970229,40.1546258197408));
#168866=CARTESIAN_POINT('Ctrl Pts',(13.1486970054272,-61.5634145183986,
40.1563626808798));
#168867=CARTESIAN_POINT('Ctrl Pts',(13.1399214696215,-61.5661391177411,
40.1576937882008));
#168868=CARTESIAN_POINT('Ctrl Pts',(13.1310016901029,-61.5686148699002,
40.1585906813668));
#168869=CARTESIAN_POINT('Ctrl Pts',(13.1265418003436,-61.5698527459797,
40.1590391279498));
#168870=CARTESIAN_POINT('Ctrl Pts',(13.1220458496817,-61.5710284103839,
40.1593790209175));
#168871=CARTESIAN_POINT('Ctrl Pts',(13.1175170363402,-61.5721388765028,
40.1596068022931));
#168872=CARTESIAN_POINT('Ctrl Pts',(13.1129882229987,-61.5732493426217,
40.1598345836687));
#168873=CARTESIAN_POINT('Ctrl Pts',(13.1084265466226,-61.5742946087864,
40.1599502506865));
#168874=CARTESIAN_POINT('Ctrl Pts',(13.1038352065726,-61.5752716937452,
40.1599502534424));
#168875=CARTESIAN_POINT('',(13.0739701745323,-61.5816197022698,40.1599502534424));
#168876=CARTESIAN_POINT('Origin',(5.62288786856779E-15,5.84690109570509E-15,
40.1599502534424));
#168877=CARTESIAN_POINT('',(12.7383709431249,-61.4590390555209,39.8576902534424));
#168878=CARTESIAN_POINT('Ctrl Pts',(13.0739701745323,-61.5816197022698,
40.1599502534424));
#168879=CARTESIAN_POINT('Ctrl Pts',(13.0702318743176,-61.5824133495499,
40.1599502447858));
#168880=CARTESIAN_POINT('Ctrl Pts',(13.0664939028184,-61.5831581321228,
40.1598744685927));
#168881=CARTESIAN_POINT('Ctrl Pts',(13.0627583804525,-61.5838547466226,
40.1597246934279));
#168882=CARTESIAN_POINT('Ctrl Pts',(13.0411716694466,-61.5878803190635,
40.1588591777435));
#168883=CARTESIAN_POINT('Ctrl Pts',(13.0196643745814,-61.590299714431,40.155525470602));
#168884=CARTESIAN_POINT('Ctrl Pts',(12.9986523536628,-61.5912450453419,
40.1500631826381));
#168885=CARTESIAN_POINT('Ctrl Pts',(12.9901777222673,-61.5916263190447,
40.1478601162481));
#168886=CARTESIAN_POINT('Ctrl Pts',(12.9817833412911,-61.5917681516647,
40.1453112228307));
#168887=CARTESIAN_POINT('Ctrl Pts',(12.9734950911672,-61.5916804171629,
40.1424401896328));
#168888=CARTESIAN_POINT('Ctrl Pts',(12.9704372300723,-61.5916480484584,
40.1413809526905));
#168889=CARTESIAN_POINT('Ctrl Pts',(12.9673939164349,-61.5915843445341,
40.1402777640511));
#168890=CARTESIAN_POINT('Ctrl Pts',(12.9643665007549,-61.5914897592007,
40.1391317641987));
#168891=CARTESIAN_POINT('Ctrl Pts',(12.9586900963549,-61.5913124117004,
40.1369830144753));
#168892=CARTESIAN_POINT('Ctrl Pts',(12.95306958321,-61.5910264967402,40.1346837565849));
#168893=CARTESIAN_POINT('Ctrl Pts',(12.9475138635631,-61.5906350058491,
40.1322415082996));
#168894=CARTESIAN_POINT('Ctrl Pts',(12.9280688447993,-61.58926478773,40.1236936393008));
#168895=CARTESIAN_POINT('Ctrl Pts',(12.9094175454591,-61.586601260073,40.113394140767));
#168896=CARTESIAN_POINT('Ctrl Pts',(12.8919416545041,-61.5827727094485,
40.101665321223));
#168897=CARTESIAN_POINT('Ctrl Pts',(12.8832037090265,-61.5808584341363,
40.095800911451));
#168898=CARTESIAN_POINT('Ctrl Pts',(12.8747596158555,-61.5786529040703,
40.0895791707949));
#168899=CARTESIAN_POINT('Ctrl Pts',(12.8666570879116,-61.5761721637749,
40.0830403822906));
#168900=CARTESIAN_POINT('Ctrl Pts',(12.8626058239396,-61.5749317936272,
40.0797709880385));
#168901=CARTESIAN_POINT('Ctrl Pts',(12.8586399512977,-61.5736226210372,
40.0764223317514));
#168902=CARTESIAN_POINT('Ctrl Pts',(12.8547654342064,-61.5722466520922,
40.0729994484778));
#168903=CARTESIAN_POINT('Ctrl Pts',(12.8508909171151,-61.5708706831472,
40.0695765652042));
#168904=CARTESIAN_POINT('Ctrl Pts',(12.8471078617859,-61.5694278436302,
40.0660793733488));
#168905=CARTESIAN_POINT('Ctrl Pts',(12.8434220158074,-61.5679202927796,
40.0625130768817));
#168906=CARTESIAN_POINT('Ctrl Pts',(12.8433905832605,-61.5679074365281,
40.0624826638418));
#168907=CARTESIAN_POINT('Ctrl Pts',(12.8433591578474,-61.5678945756943,
40.0624522459912));
#168908=CARTESIAN_POINT('Ctrl Pts',(12.8433277395707,-61.5678817102796,
40.0624218233329));
#168909=CARTESIAN_POINT('Ctrl Pts',(12.8272819669698,-61.561311155148,40.0468845275908));
#168910=CARTESIAN_POINT('Ctrl Pts',(12.8130163727087,-61.5536499750616,
40.0302263329259));
#168911=CARTESIAN_POINT('Ctrl Pts',(12.8005145062075,-61.5450979154855,
40.0127515884777));
#168912=CARTESIAN_POINT('Ctrl Pts',(12.7875898348827,-61.5362566309333,
39.9946858597759));
#168913=CARTESIAN_POINT('Ctrl Pts',(12.7765497640396,-61.5264624086177,
39.9757460620546));
#168914=CARTESIAN_POINT('Ctrl Pts',(12.7674219834083,-61.5159109908837,
39.9562444559197));
#168915=CARTESIAN_POINT('Ctrl Pts',(12.7584678323715,-61.5055602833174,
39.9371138113689));
#168916=CARTESIAN_POINT('Ctrl Pts',(12.7513538295754,-61.4944799879548,
39.9174410654441));
#168917=CARTESIAN_POINT('Ctrl Pts',(12.7461528104596,-61.4828443590724,
39.8975196504242));
#168918=CARTESIAN_POINT('Ctrl Pts',(12.742707317634,-61.4751361628628,39.884322411384));
#168919=CARTESIAN_POINT('Ctrl Pts',(12.7401023057314,-61.4671840587593,
39.8710160447164));
#168920=CARTESIAN_POINT('Ctrl Pts',(12.7383709431249,-61.4590390555209,
39.8576902534424));
#168921=CARTESIAN_POINT('',(12.664289321014,-61.1105274371641,39.2875012672119));
#168922=CARTESIAN_POINT('',(12.7383709431249,-61.4590390555209,39.8576902534424));
#168923=CARTESIAN_POINT('',(6.8397366303024,-62.0330459552233,39.2875012672119));
#168924=CARTESIAN_POINT('Origin',(5.53234440788222E-15,0.,39.2875012672119));
#168925=CARTESIAN_POINT('',(6.87697683366544,-62.3873926810691,39.8576902534424));
#168926=CARTESIAN_POINT('',(6.8397366303024,-62.0330459552233,39.2875012672119));
#168927=CARTESIAN_POINT('',(6.59568250079865,-62.6076796697354,40.1599502534424));
#168928=CARTESIAN_POINT('Ctrl Pts',(6.87697683366544,-62.3873926810691,
39.8576902534424));
#168929=CARTESIAN_POINT('Ctrl Pts',(6.87826302285563,-62.3996312165467,
39.8773836120355));
#168930=CARTESIAN_POINT('Ctrl Pts',(6.87760542309009,-62.4120334591682,
39.8969946442113));
#168931=CARTESIAN_POINT('Ctrl Pts',(6.87506472947593,-62.4244204973379,
39.9162525288213));
#168932=CARTESIAN_POINT('Ctrl Pts',(6.87247298342313,-62.4370564393905,
39.9358973794026));
#168933=CARTESIAN_POINT('Ctrl Pts',(6.86792184690411,-62.4496774784054,
39.9551762199694));
#168934=CARTESIAN_POINT('Ctrl Pts',(6.86142424476998,-62.4621080448309,
39.9738152034189));
#168935=CARTESIAN_POINT('Ctrl Pts',(6.85517906858854,-62.4740556950194,
39.991730079258));
#168936=CARTESIAN_POINT('Ctrl Pts',(6.84713544261344,-62.4858282202819,
40.0090551158049));
#168937=CARTESIAN_POINT('Ctrl Pts',(6.83725958233785,-62.4972698477072,
40.0255394551454));
#168938=CARTESIAN_POINT('Ctrl Pts',(6.82967328917275,-62.5060589088635,
40.0382021526098));
#168939=CARTESIAN_POINT('Ctrl Pts',(6.82100495425341,-62.5146528151136,
40.0503687782099));
#168940=CARTESIAN_POINT('Ctrl Pts',(6.8112212579066,-62.5229765487297,40.0619155352442));
#168941=CARTESIAN_POINT('Ctrl Pts',(6.8111956165833,-62.5229983637511,40.0619457972351));
#168942=CARTESIAN_POINT('Ctrl Pts',(6.8111699667641,-62.5230201768492,40.0619760547305));
#168943=CARTESIAN_POINT('Ctrl Pts',(6.81114430845137,-62.5230419880217,
40.0620063077269));
#168944=CARTESIAN_POINT('Ctrl Pts',(6.80839321554227,-62.5253805892671,
40.06525004417));
#168945=CARTESIAN_POINT('Ctrl Pts',(6.80554511475049,-62.5276952632611,
40.0684393223556));
#168946=CARTESIAN_POINT('Ctrl Pts',(6.80260378684096,-62.5299828381018,
40.0715697951759));
#168947=CARTESIAN_POINT('Ctrl Pts',(6.78623596579486,-62.5427126719642,
40.0889901646441));
#168948=CARTESIAN_POINT('Ctrl Pts',(6.7669842911974,-62.5546072354152,40.104596309828));
#168949=CARTESIAN_POINT('Ctrl Pts',(6.74555473733804,-62.5651294462146,
40.1176634650772));
#168950=CARTESIAN_POINT('Ctrl Pts',(6.7359368568061,-62.5698519601346,40.1235281853091));
#168951=CARTESIAN_POINT('Ctrl Pts',(6.72588021343273,-62.5742983919741,
40.1288820140933));
#168952=CARTESIAN_POINT('Ctrl Pts',(6.71544740276754,-62.5784220664834,
40.1336621774101));
#168953=CARTESIAN_POINT('Ctrl Pts',(6.7109134443649,-62.580214159649,40.1357395717319));
#168954=CARTESIAN_POINT('Ctrl Pts',(6.70630855228273,-62.5819451239082,
40.1377083672883));
#168955=CARTESIAN_POINT('Ctrl Pts',(6.70163794008953,-62.5836110216378,
40.1395632548791));
#168956=CARTESIAN_POINT('Ctrl Pts',(6.68529079741335,-62.5894416636913,
40.146055361447));
#168957=CARTESIAN_POINT('Ctrl Pts',(6.66813858303382,-62.5944752375494,
40.1511520974629));
#168958=CARTESIAN_POINT('Ctrl Pts',(6.65040483057317,-62.5985429352696,
40.1546258197408));
#168959=CARTESIAN_POINT('Ctrl Pts',(6.64153795434284,-62.6005767841297,
40.1563626808798));
#168960=CARTESIAN_POINT('Ctrl Pts',(6.63252569365821,-62.6023691645599,
40.1576937882008));
#168961=CARTESIAN_POINT('Ctrl Pts',(6.62339599105649,-62.6038989834438,
40.1585906813668));
#168962=CARTESIAN_POINT('Ctrl Pts',(6.61883113975563,-62.6046638928858,
40.1590391279498));
#168963=CARTESIAN_POINT('Ctrl Pts',(6.61423692798836,-62.6053631620637,
40.1593790209175));
#168964=CARTESIAN_POINT('Ctrl Pts',(6.60961684864331,-62.605994155034,40.1596068022931));
#168965=CARTESIAN_POINT('Ctrl Pts',(6.60499676929825,-62.6066251480043,
40.1598345836687));
#168966=CARTESIAN_POINT('Ctrl Pts',(6.6003508221967,-62.60718786307,40.1599502506864));
#168967=CARTESIAN_POINT('Ctrl Pts',(6.59568250079866,-62.6076796697354,
40.1599502534424));
#168968=CARTESIAN_POINT('',(6.56531752495282,-62.6108711573006,40.1599502534424));
#168969=CARTESIAN_POINT('Origin',(5.63895492999586E-15,5.84944586823703E-15,
40.1599502534424));
#168970=CARTESIAN_POINT('',(6.24436990788039,-62.4538823482276,39.8576902534424));
#168971=CARTESIAN_POINT('Ctrl Pts',(6.56531752495282,-62.6108711573006,
40.1599502534424));
#168972=CARTESIAN_POINT('Ctrl Pts',(6.56151674480723,-62.611269698121,40.1599502447857));
#168973=CARTESIAN_POINT('Ctrl Pts',(6.55772139932922,-62.6116196762807,
40.1598744685927));
#168974=CARTESIAN_POINT('Ctrl Pts',(6.55393352450261,-62.6119220062409,
40.1597246934279));
#168975=CARTESIAN_POINT('Ctrl Pts',(6.53204428085673,-62.6136691004464,
40.1588591777435));
#168976=CARTESIAN_POINT('Ctrl Pts',(6.51040190952292,-62.6138271176315,
40.1555254706019));
#168977=CARTESIAN_POINT('Ctrl Pts',(6.48940618066564,-62.612570915664,40.1500631826377));
#168978=CARTESIAN_POINT('Ctrl Pts',(6.48093812023387,-62.612064260513,40.1478601162478));
#168979=CARTESIAN_POINT('Ctrl Pts',(6.4725748990096,-62.6113278644156,40.1453112228305));
#168980=CARTESIAN_POINT('Ctrl Pts',(6.46434122354013,-62.610374252484,40.1424401896328));
#168981=CARTESIAN_POINT('Ctrl Pts',(6.46130349717921,-62.6100224275775,
40.1413809526906));
#168982=CARTESIAN_POINT('Ctrl Pts',(6.45828351400566,-62.6096409597322,
40.1402777640512));
#168983=CARTESIAN_POINT('Ctrl Pts',(6.45528256968506,-62.6092304414384,
40.1391317641987));
#168984=CARTESIAN_POINT('Ctrl Pts',(6.44965579908394,-62.6084607196375,
40.1369830144753));
#168985=CARTESIAN_POINT('Ctrl Pts',(6.44409596194954,-62.6075888673476,
40.1346837565849));
#168986=CARTESIAN_POINT('Ctrl Pts',(6.43861159905749,-62.6066187902474,
40.1322415082996));
#168987=CARTESIAN_POINT('Ctrl Pts',(6.41941632893531,-62.6032235203971,
40.1236936393009));
#168988=CARTESIAN_POINT('Ctrl Pts',(6.40114561781732,-62.5986249921653,
40.113394140767));
#168989=CARTESIAN_POINT('Ctrl Pts',(6.38416565413474,-62.5929906867159,
40.101665321223));
#168990=CARTESIAN_POINT('Ctrl Pts',(6.37567567229345,-62.5901735339912,
40.095800911451));
#168991=CARTESIAN_POINT('Ctrl Pts',(6.36750837741685,-62.5870974379668,
40.0895791707949));
#168992=CARTESIAN_POINT('Ctrl Pts',(6.35970954393957,-62.5837833426318,
40.0830403822906));
#168993=CARTESIAN_POINT('Ctrl Pts',(6.35581012720093,-62.5821262949642,
40.0797709880385));
#168994=CARTESIAN_POINT('Ctrl Pts',(6.35200282582339,-62.5804097475859,
40.0764223317514));
#168995=CARTESIAN_POINT('Ctrl Pts',(6.34829336166144,-62.5786363190253,
40.0729994484778));
#168996=CARTESIAN_POINT('Ctrl Pts',(6.34458389749948,-62.5768628904647,
40.0695765652042));
#168997=CARTESIAN_POINT('Ctrl Pts',(6.3409723839406,-62.5750325180135,40.0660793733488));
#168998=CARTESIAN_POINT('Ctrl Pts',(6.33746431138575,-62.5731479498682,
40.0625130768817));
#168999=CARTESIAN_POINT('Ctrl Pts',(6.3374343948739,-62.5731318784488,40.0624826638418));
#169000=CARTESIAN_POINT('Ctrl Pts',(6.33740448593562,-62.5731158032179,
40.0624522459912));
#169001=CARTESIAN_POINT('Ctrl Pts',(6.33737458457357,-62.5730997241771,
40.0624218233329));
#169002=CARTESIAN_POINT('Ctrl Pts',(6.32210352242537,-62.5648879232825,
40.0468845275917));
#169003=CARTESIAN_POINT('Ctrl Pts',(6.30871688796422,-62.5557775512971,
40.0302263329276));
#169004=CARTESIAN_POINT('Ctrl Pts',(6.29717744164146,-62.5459655399053,
40.0127515884805));
#169005=CARTESIAN_POINT('Ctrl Pts',(6.28524773890653,-62.5358216928038,
39.9946858597798));
#169006=CARTESIAN_POINT('Ctrl Pts',(6.27529192173438,-62.524927122624,39.9757460620596));
#169007=CARTESIAN_POINT('Ctrl Pts',(6.26731706752152,-62.5134793937786,
39.9562444559258));
#169008=CARTESIAN_POINT('Ctrl Pts',(6.25949391181652,-62.5022494248242,
39.9371138113761));
#169009=CARTESIAN_POINT('Ctrl Pts',(6.25357708651871,-62.4904862126997,
39.9174410654523));
#169010=CARTESIAN_POINT('Ctrl Pts',(6.24962081353557,-62.4783706704748,
39.8975196504334));
#169011=CARTESIAN_POINT('Ctrl Pts',(6.2469999213836,-62.4703445484985,39.8843224113901));
#169012=CARTESIAN_POINT('Ctrl Pts',(6.24524040122982,-62.4621637089605,
39.8710160447195));
#169013=CARTESIAN_POINT('Ctrl Pts',(6.2443699078804,-62.4538823482276,39.8576902534424));
#169014=CARTESIAN_POINT('',(6.20712349654444,-62.0995362748659,39.2875012672119));
#169015=CARTESIAN_POINT('',(6.24436990788039,-62.4538823482276,39.8576902534424));
#169016=CARTESIAN_POINT('',(0.318048871876918,-62.4081695979768,39.2875012672119));
#169017=CARTESIAN_POINT('Origin',(5.53234440788222E-15,0.,39.2875012672119));
#169018=CARTESIAN_POINT('',(0.318045750792831,-62.7644678366119,39.8576902534424));
#169019=CARTESIAN_POINT('',(0.318048871876917,-62.4081695979768,39.2875012672119));
#169020=CARTESIAN_POINT('',(0.0152661173106527,-62.9541448057648,40.1599502534424));
#169021=CARTESIAN_POINT('Ctrl Pts',(0.318045750792832,-62.7644678366119,
39.8576902534424));
#169022=CARTESIAN_POINT('Ctrl Pts',(0.318045618797918,-62.77677377149,39.8773836120337));
#169023=CARTESIAN_POINT('Ctrl Pts',(0.316095234070707,-62.7890393354348,
39.8969946442078));
#169024=CARTESIAN_POINT('Ctrl Pts',(0.312273660578351,-62.8010929413131,
39.9162525288161));
#169025=CARTESIAN_POINT('Ctrl Pts',(0.3083752967776,-62.8133887511198,39.9358973793957));
#169026=CARTESIAN_POINT('Ctrl Pts',(0.302529834048607,-62.825464927455,
39.9551762199608));
#169027=CARTESIAN_POINT('Ctrl Pts',(0.294768478454255,-62.83714821357,39.9738152034088));
#169028=CARTESIAN_POINT('Ctrl Pts',(0.287308644488887,-62.8483776146106,
39.9917300792465));
#169029=CARTESIAN_POINT('Ctrl Pts',(0.278078518365733,-62.8592448608849,
40.009055115792));
#169030=CARTESIAN_POINT('Ctrl Pts',(0.267060783356072,-62.8695915013792,
40.0255394551315));
#169031=CARTESIAN_POINT('Ctrl Pts',(0.258597341640148,-62.8775394315757,
40.0382021526009));
#169032=CARTESIAN_POINT('Ctrl Pts',(0.249078184949622,-62.8851801717828,
40.0503687782056));
#169033=CARTESIAN_POINT('Ctrl Pts',(0.238478017627655,-62.8924356323738,
40.0619155352442));
#169034=CARTESIAN_POINT('Ctrl Pts',(0.238450236479546,-62.892454647642,
40.0619457972351));
#169035=CARTESIAN_POINT('Ctrl Pts',(0.238422447083121,-62.8924736601095,
40.0619760547305));
#169036=CARTESIAN_POINT('Ctrl Pts',(0.238394649440958,-62.8924926697742,
40.0620063077269));
#169037=CARTESIAN_POINT('Ctrl Pts',(0.235414176912292,-62.8945308924032,
40.06525004417));
